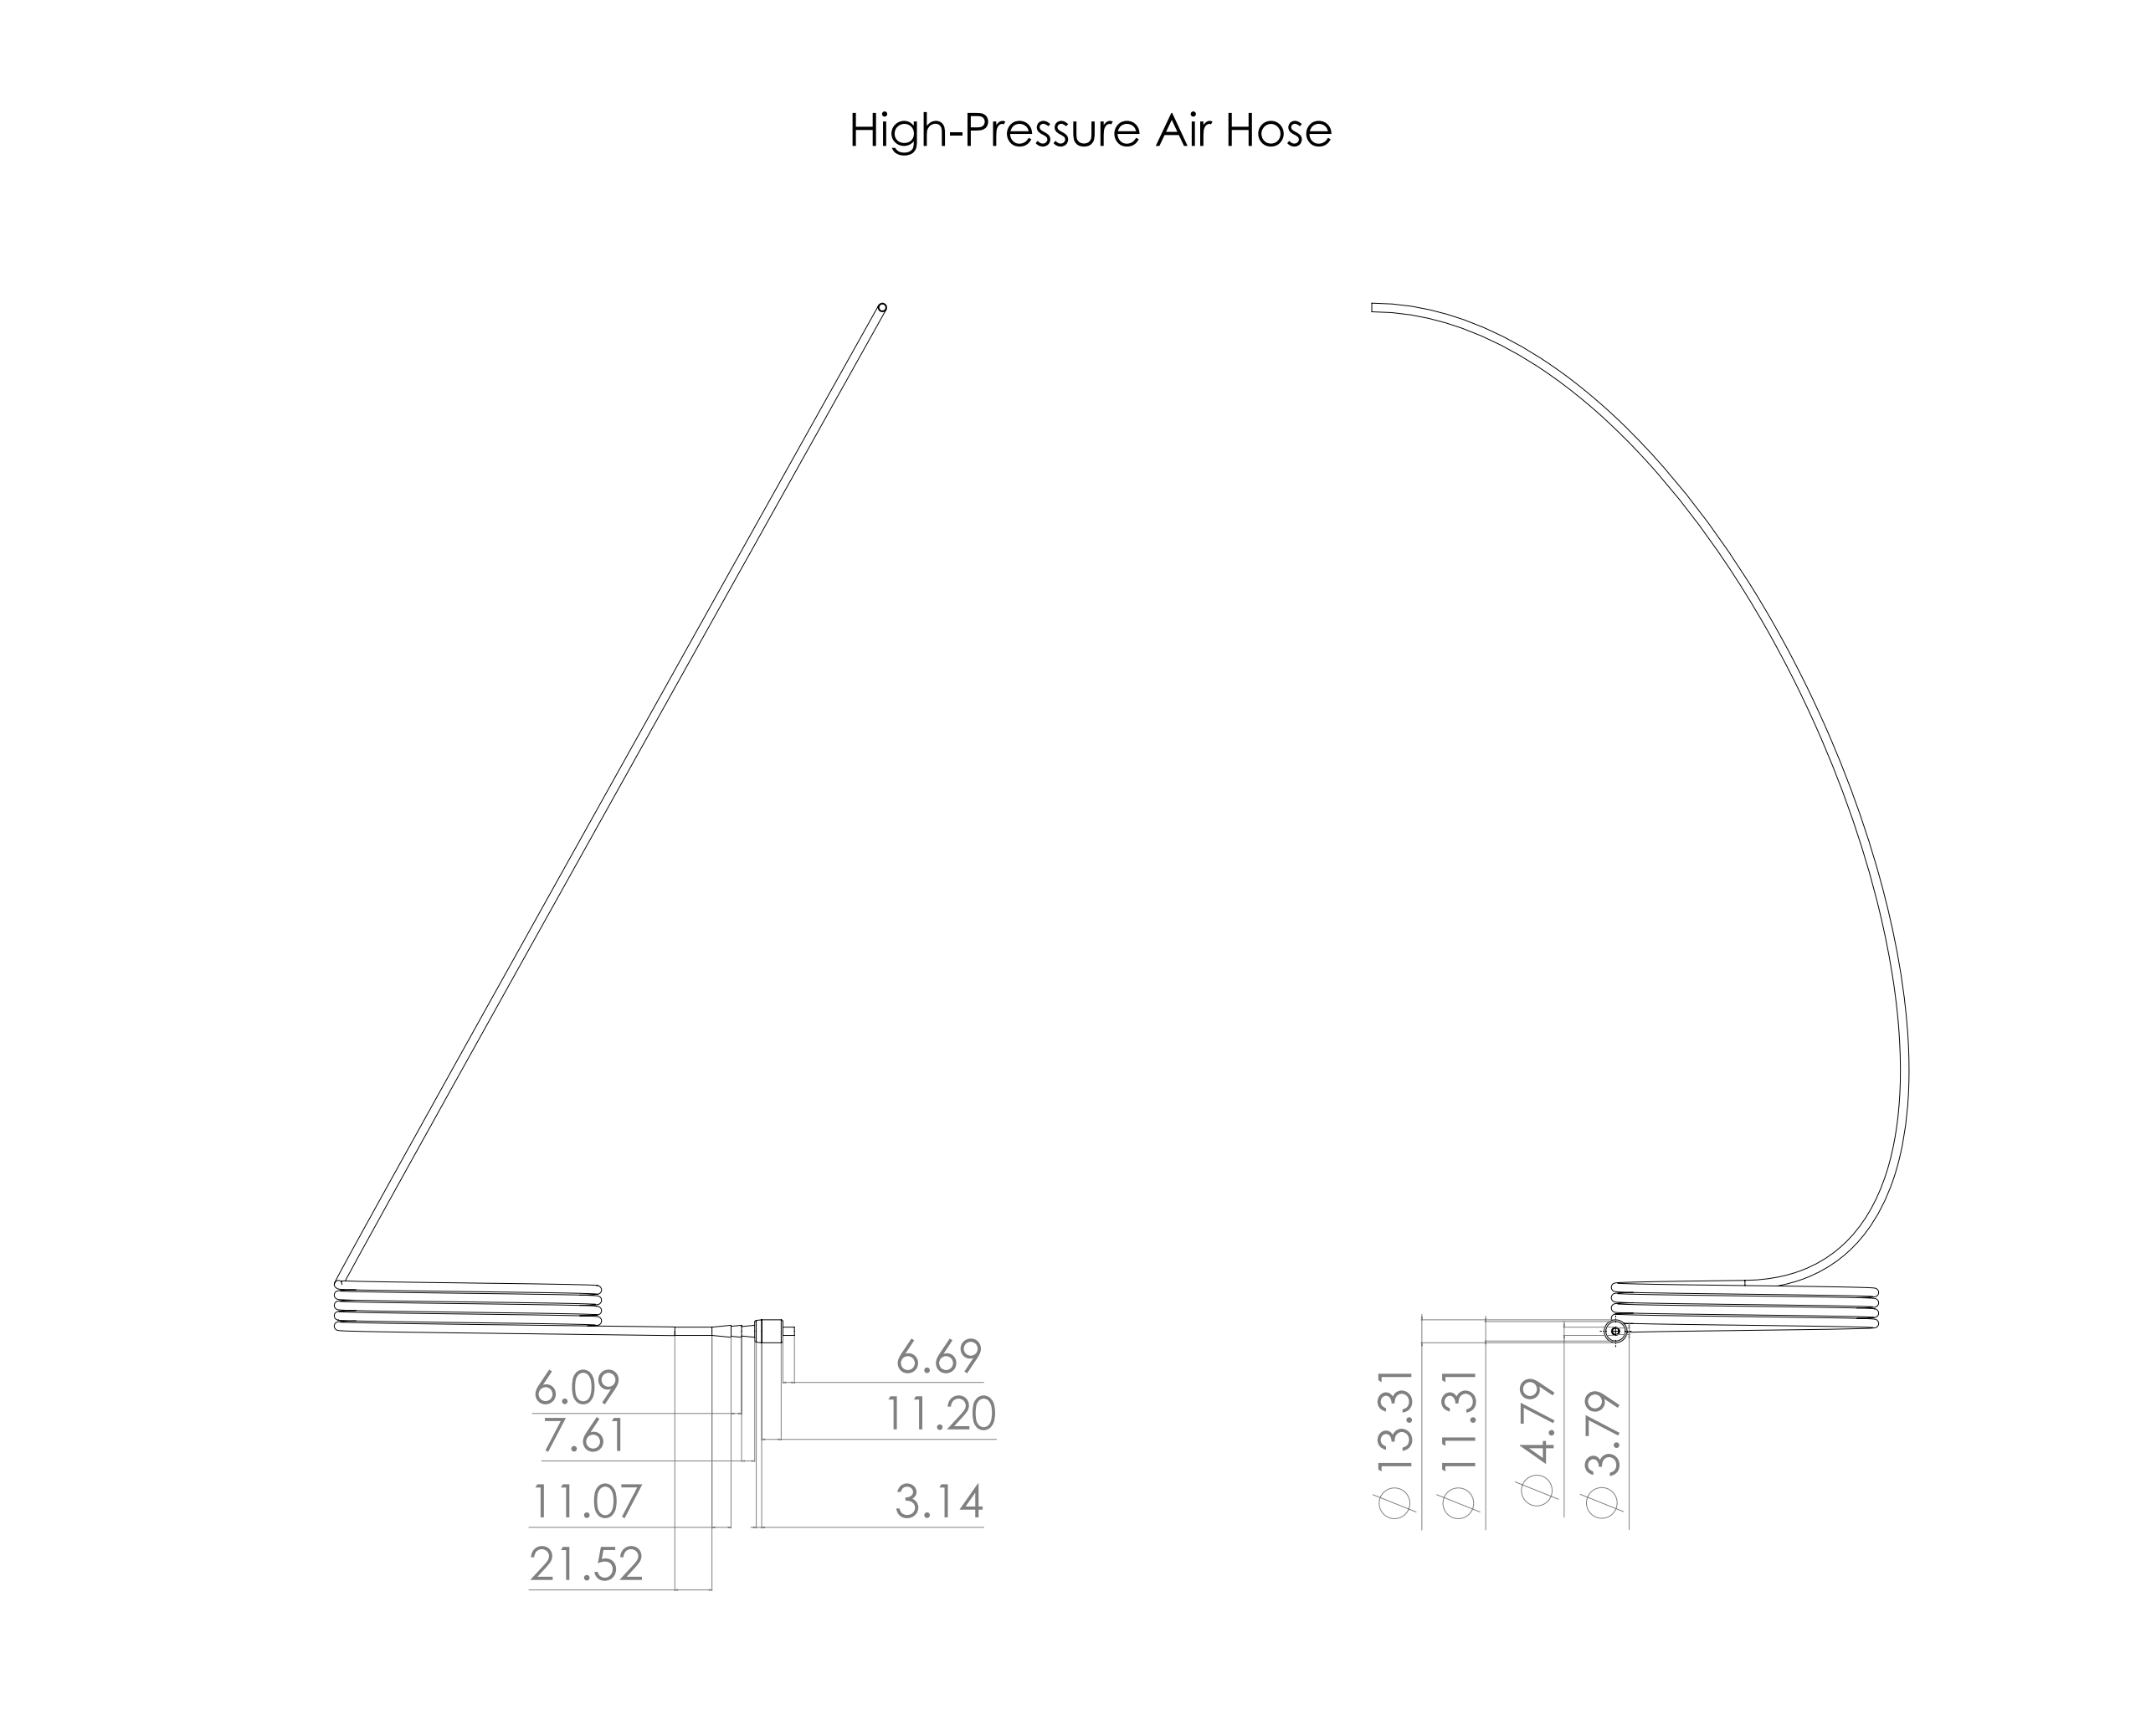
ISO-10303-21;
HEADER;
FILE_DESCRIPTION (('STEP AP214'),
    '1' );
FILE_NAME ('High-Pressure Air Hose.step',
    '2026-10-25T20:52:49',
    ( '' ),
    ( '' ),
    'SwSTEP 2.0',
    'SolidWorks 2025',
    '' );
FILE_SCHEMA (( 'AUTOMOTIVE_DESIGN' ));
ENDSEC;

DATA;
#1=CARTESIAN_POINT ( 'NONE',  ( -113.6132551642233466, -295.8660902273127817, -261.0439986488574391 ) ) ;
#2=CARTESIAN_POINT ( 'NONE',  ( -21.69829453939080111, -272.4952783879842286, -198.0198581616166962 ) ) ;
#3=CARTESIAN_POINT ( 'NONE',  ( -77.14607672046975040, -275.6695791045739270, -333.3258523244866751 ) ) ;
#4=CARTESIAN_POINT ( 'NONE',  ( -96.50722556860337420, -298.4744652489187047, -226.7430298893199279 ) ) ;
#5=CARTESIAN_POINT ( 'NONE',  ( 35.29261755122405475, -294.8217676056252117, -258.4658906454228031 ) ) ;
#7=CARTESIAN_POINT ( 'NONE',  ( 17.20777486049739124, -295.0510334597752831, -319.1340501124739717 ) ) ;
#10=CARTESIAN_POINT ( 'NONE',  ( 23.39288443123379579, -284.9668621146994951, -225.7548735365318748 ) ) ;
#11=CARTESIAN_POINT ( 'NONE',  ( -84.47810206200919936, -295.7221423797171838, -326.1693894271719500 ) ) ;
#12=CARTESIAN_POINT ( 'NONE',  ( -83.27587881292458860, -285.4425543175578923, -208.4961557201596918 ) ) ;
#14=CARTESIAN_POINT ( 'NONE',  ( 24.12276456990134577, -287.8361799259163263, -316.7061702643556487 ) ) ;
#15=CARTESIAN_POINT ( 'NONE',  ( -83.16459577638245548, -297.6555613683490265, -330.2488683299737886 ) ) ;
#16=CARTESIAN_POINT ( 'NONE',  ( 12.16221636192367228, -290.7420802479286976, -214.1725176534357615 ) ) ;
#17=CARTESIAN_POINT ( 'NONE',  ( -48.08606759839130973, -279.1160864900698471, -194.2237662435092886 ) ) ;
#18=CARTESIAN_POINT ( 'NONE',  ( -110.4683760289727132, -293.8380690714490129, -287.0191576251351080 ) ) ;
#20=CARTESIAN_POINT ( 'NONE',  ( 26.72141337091415991, -285.8585362577462661, -234.4374339655554991 ) ) ;
#21=DIRECTION ( 'NONE',  ( -1.000000000000000000, -0.000000000000000000, -0.000000000000000000 ) ) ;
#23=CARTESIAN_POINT ( 'NONE',  ( -111.0120785373717354, -298.2093386174307170, -265.9889607955867632 ) ) ;
#24=CARTESIAN_POINT ( 'NONE',  ( -9.095926160855869469, -281.8396501160608523, -199.3626493647371376 ) ) ;
#25=CARTESIAN_POINT ( 'NONE',  ( -109.2360963732521952, -294.8641011722828580, -247.6139534407837743 ) ) ;
#26=CARTESIAN_POINT ( 'NONE',  ( 24.14595339631129534, -281.7647060850542289, -309.8413200465337241 ) ) ;
#27=CARTESIAN_POINT ( 'NONE',  ( -106.5142501024570265, -297.1531912002984086, -236.5357083837597827 ) ) ;
#29=CARTESIAN_POINT ( 'NONE',  ( -110.4578234273896271, -280.7667899122553763, -253.6568320815989921 ) ) ;
#30=CARTESIAN_POINT ( 'NONE',  ( -93.78727130258138800, -296.2704692607680386, -223.6800016881232693 ) ) ;
#33=CARTESIAN_POINT ( 'NONE',  ( -91.92744132223316456, -285.8159430608695288, -321.2751991526628785 ) ) ;
#35=CARTESIAN_POINT ( 'NONE',  ( -110.4542110544635705, -294.2666405000204577, -253.6410175316879361 ) ) ;
#36=CARTESIAN_POINT ( 'NONE',  ( 16.83410871617971338, -275.5019898621288235, -324.9252248568274126 ) ) ;
#37=CARTESIAN_POINT ( 'NONE',  ( -6.039705354571541562, -292.3087031825515965, -204.3989839164147782 ) ) ;
#38=CARTESIAN_POINT ( 'NONE',  ( 33.63237012736230724, -283.3319559697839054, -290.1951570289018605 ) ) ;
#39=CARTESIAN_POINT ( 'NONE',  ( 33.67317559943808192, -277.4154469211121636, -290.4904342910287482 ) ) ;
#40=CARTESIAN_POINT ( 'NONE',  ( -68.83699650705307249, -285.0594432950156829, -339.7618826965099856 ) ) ;
#41=CARTESIAN_POINT ( 'NONE',  ( 30.69690168102419747, -280.7137460309204471, -297.8907232790041348 ) ) ;
#42=CARTESIAN_POINT ( 'NONE',  ( -110.7162897014109433, -280.3529109521358009, -285.8907753398488580 ) ) ;
#43=CARTESIAN_POINT ( 'NONE',  ( -113.8629036840343218, -272.8260555190163927, -261.7875883216721036 ) ) ;
#44=CARTESIAN_POINT ( 'NONE',  ( 36.88505382238304264, -275.6425748523263906, -290.8892655207978351 ) ) ;
#45=CARTESIAN_POINT ( 'NONE',  ( 22.49833801616120255, -296.0810694518352193, -314.6384715069982576 ) ) ;
#49=CARTESIAN_POINT ( 'NONE',  ( -61.22503046524085590, -293.4984592147682747, -342.3179306570231688 ) ) ;
#50=CARTESIAN_POINT ( 'NONE',  ( -56.87203779738695175, -273.3011920805299724, -199.9055576269083190 ) ) ;
#51=CARTESIAN_POINT ( 'NONE',  ( -39.21425765019228038, -293.5492008878248384, -194.0645109205592576 ) ) ;
#52=CARTESIAN_POINT ( 'NONE',  ( -72.08107566293803359, -300.1233781216987495, -198.2974183793908196 ) ) ;
#53=CARTESIAN_POINT ( 'NONE',  ( -22.28692340252414539, -293.4457659912081908, -195.1980702719413614 ) ) ;
#54=CARTESIAN_POINT ( 'NONE',  ( 17.36828252781073800, -290.2692810089828868, -321.4942518745497182 ) ) ;
#55=CARTESIAN_POINT ( 'NONE',  ( -112.2266234623324124, -276.5486602746883023, -270.6195867653905793 ) ) ;
#56=CARTESIAN_POINT ( 'NONE',  ( -81.65742486183103210, -279.5809590698107172, -330.1727450829594659 ) ) ;
#57=CARTESIAN_POINT ( 'NONE',  ( 35.17272386656721750, -291.8502700334059909, -287.2389789927554489 ) ) ;
#58=CARTESIAN_POINT ( 'NONE',  ( 33.44209198229489743, -283.7601780698271341, -297.3788945958802969 ) ) ;
#59=CARTESIAN_POINT ( 'NONE',  ( -109.8060437348913467, -283.3224215553644285, -281.7842631819470398 ) ) ;
#60=ORIENTED_EDGE ( 'NONE', *, *, #32885, .T. ) ;
#61=CARTESIAN_POINT ( 'NONE',  ( -71.42250952254038054, -283.1821142129608120, -334.9411916729687277 ) ) ;
#62=CARTESIAN_POINT ( 'NONE',  ( -28.27524738754997813, -281.2441658516256098, -194.1546269278096304 ) ) ;
#63=CARTESIAN_POINT ( 'NONE',  ( -113.4234760108877538, -283.4592184142248357, -261.4407986698293485 ) ) ;
#64=CARTESIAN_POINT ( 'NONE',  ( -109.5114376524103363, -279.1602184646021101, -296.6766189074363638 ) ) ;
#66=CARTESIAN_POINT ( 'NONE',  ( -97.37137399137552052, -279.4367685291730368, -317.4689306191668265 ) ) ;
#68=CARTESIAN_POINT ( 'NONE',  ( -6.941161984400275209, -297.1233781216987495, -333.4151289067050357 ) ) ;
#71=CARTESIAN_POINT ( 'NONE',  ( -93.35509533216730915, -299.2464325822394926, -220.4862725388631191 ) ) ;
#73=CARTESIAN_POINT ( 'NONE',  ( -88.23497865206087454, -275.7892183208580263, -324.9662551183911319 ) ) ;
#74=CARTESIAN_POINT ( 'NONE',  ( -102.3605472477040337, -292.8335325276641470, -230.9337581368000087 ) ) ;
#75=CARTESIAN_POINT ( 'NONE',  ( 34.31805428248770795, -292.7103970009527529, -255.9121641687935949 ) ) ;
#76=CARTESIAN_POINT ( 'NONE',  ( -96.34789938153127764, -289.3946153186523702, -319.7555901667715261 ) ) ;
#78=CARTESIAN_POINT ( 'NONE',  ( 36.88326735793300060, -292.3562425583122035, -288.5613484753777129 ) ) ;
#79=CARTESIAN_POINT ( 'NONE',  ( -33.17331374697837987, -284.5052435883285966, -196.6285636872405860 ) ) ;
#80=CARTESIAN_POINT ( 'NONE',  ( -69.57500681174269630, -293.4837748164715094, -203.4749671060159528 ) ) ;
#81=CARTESIAN_POINT ( 'NONE',  ( 22.22138339417639230, -283.4657779623778993, -313.4347628960813381 ) ) ;
#82=CARTESIAN_POINT ( 'NONE',  ( -28.99082608718071796, -289.8901462222868872, -346.7236095928074064 ) ) ;
#83=CARTESIAN_POINT ( 'NONE',  ( 34.39346676443356188, -281.8609718709653862, -256.4368729998031426 ) ) ;
#84=CARTESIAN_POINT ( 'NONE',  ( 39.20951696572362977, -292.3824562929385706, -273.1753459359540557 ) ) ;
#85=CARTESIAN_POINT ( 'NONE',  ( -4.393016225146153531, -289.4317384794202326, -339.7912944455955540 ) ) ;
#86=CARTESIAN_POINT ( 'NONE',  ( 37.65823291392757000, -287.8290301222977519, -253.1405899415904912 ) ) ;
#87=CARTESIAN_POINT ( 'NONE',  ( -52.09100773288315622, -286.0247242745892322, -198.8666571505329728 ) ) ;
#90=CARTESIAN_POINT ( 'NONE',  ( 3.580403759654407825, -296.3688474698320192, -334.1856371305267430 ) ) ;
#91=CARTESIAN_POINT ( 'NONE',  ( -113.1662103178394432, -295.1037629167083196, -280.9449385996212527 ) ) ;
#93=CARTESIAN_POINT ( 'NONE',  ( -83.57703501779413102, -278.4588845934780466, -213.5002235206053740 ) ) ;
#94=CARTESIAN_POINT ( 'NONE',  ( -113.8008141857499993, -272.1671345119243028, -261.7861089057840900 ) ) ;
#95=CARTESIAN_POINT ( 'NONE',  ( -103.3981541237931054, -294.5919941891141889, -303.1453271309203501 ) ) ;
#96=CARTESIAN_POINT ( 'NONE',  ( 35.36480375133581333, -277.1321324331269693, -256.5141577024394337 ) ) ;
#97=CARTESIAN_POINT ( 'NONE',  ( -54.47399014668751249, -271.9692736385993044, -198.1298912440302331 ) ) ;
#98=CARTESIAN_POINT ( 'NONE',  ( 29.09142378860511258, -294.3365518058123484, -239.0359238687793777 ) ) ;
#99=CARTESIAN_POINT ( 'NONE',  ( -75.80859898051943446, -296.6581450815154994, -332.8264140846681016 ) ) ;
#101=CARTESIAN_POINT ( 'NONE',  ( -85.24696079806301441, -293.7120025854050596, -328.2844675371921994 ) ) ;
#102=CARTESIAN_POINT ( 'NONE',  ( -114.1802237732302245, -273.3548555386022372, -270.3713173946429720 ) ) ;
#103=CARTESIAN_POINT ( 'NONE',  ( -94.45286519521168600, -275.2254758110098010, -221.7273418318577569 ) ) ;
#104=CARTESIAN_POINT ( 'NONE',  ( -108.8900272069156472, -291.2871953198740016, -286.0477213144812936 ) ) ;
#105=CARTESIAN_POINT ( 'NONE',  ( -4.323302397459051427, -294.9377782480969472, -335.5047827706411567 ) ) ;
#106=CARTESIAN_POINT ( 'NONE',  ( -112.5882073356291926, -280.4803416563776182, -274.4070978670125669 ) ) ;
#107=CARTESIAN_POINT ( 'NONE',  ( -108.0504587551557307, -277.6107128976585159, -241.1452023711554489 ) ) ;
#108=CARTESIAN_POINT ( 'NONE',  ( -33.07270939256004993, -282.3483276930217585, -347.1537153405075173 ) ) ;
#109=CARTESIAN_POINT ( 'NONE',  ( 15.96235870874075324, -274.1327303341880679, -214.9355814682232904 ) ) ;
#110=CARTESIAN_POINT ( 'NONE',  ( -96.18649800141388084, -277.6093990147008412, -221.9287466249451199 ) ) ;
#111=CARTESIAN_POINT ( 'NONE',  ( -61.43528157839729431, -277.7399057781236706, -199.1056149990290294 ) ) ;
#112=CARTESIAN_POINT ( 'NONE',  ( -67.00311722930408109, -296.3398741006864157, -203.1056652694137199 ) ) ;
#113=CARTESIAN_POINT ( 'NONE',  ( -33.55588428573118165, -276.0999399286864104, -195.4440965705611575 ) ) ;
#115=CARTESIAN_POINT ( 'NONE',  ( 5.580496127948171292, -290.6504686268311843, -208.4249260671794843 ) ) ;
#116=CARTESIAN_POINT ( 'NONE',  ( -112.2626902172997205, -290.3291827781827692, -288.1895695498705550 ) ) ;
#117=CARTESIAN_POINT ( 'NONE',  ( -66.84020672111827821, -275.6666780896798059, -201.2245391158463406 ) ) ;
#118=CARTESIAN_POINT ( 'NONE',  ( -41.95658063400141202, -295.9936855060223024, -195.6702128762018162 ) ) ;
#119=CARTESIAN_POINT ( 'NONE',  ( -106.5292690430238025, -284.1790909977862043, -236.9359907930603981 ) ) ;
#120=CARTESIAN_POINT ( 'NONE',  ( -37.35456021389456538, -284.0517986001094073, -195.3485413134038424 ) ) ;
#122=CARTESIAN_POINT ( 'NONE',  ( 17.04267055929170738, -291.6439787220554649, -220.9968955086508515 ) ) ;
#123=CARTESIAN_POINT ( 'NONE',  ( -62.96739064857778345, -283.8546313715036717, -200.6342915240590230 ) ) ;
#126=CARTESIAN_POINT ( 'NONE',  ( 7.902484555432940816, -290.6701741179288092, -210.5450298619024636 ) ) ;
#127=CARTESIAN_POINT ( 'NONE',  ( -89.97405692109779807, -282.2588973123018832, -325.6834086931719412 ) ) ;
#128=CARTESIAN_POINT ( 'NONE',  ( -103.8431496891660544, -279.7226268398578668, -302.4792602913342421 ) ) ;
#129=CARTESIAN_POINT ( 'NONE',  ( -65.74447246362868214, -286.8938844950662883, -199.2042825010933313 ) ) ;
#130=CARTESIAN_POINT ( 'NONE',  ( -9.493390062269362772, -286.4264726012228266, -202.8681937675485756 ) ) ;
#131=CARTESIAN_POINT ( 'NONE',  ( -94.04857214285830480, -279.3176295112319281, -317.2818740737955068 ) ) ;
#132=CARTESIAN_POINT ( 'NONE',  ( -94.07220428401220147, -280.0074554778488505, -224.1631567100062625 ) ) ;
#134=CARTESIAN_POINT ( 'NONE',  ( -96.45200547131824464, -285.9190198393021092, -316.5235751886017397 ) ) ;
#136=CARTESIAN_POINT ( 'NONE',  ( -46.12776598691637275, -297.7769461629130774, -193.8640261997899188 ) ) ;
#138=CARTESIAN_POINT ( 'NONE',  ( -23.45499506039496396, -290.8538007153030662, -343.7556936576084468 ) ) ;
#141=CARTESIAN_POINT ( 'NONE',  ( -72.02372285203398405, -285.9805209788416391, -342.4524372437778652 ) ) ;
#143=CARTESIAN_POINT ( 'NONE',  ( 35.52797234631308498, -291.6693239864514453, -248.0799319934128278 ) ) ;
#144=CARTESIAN_POINT ( 'NONE',  ( -9.246811333089969054, -287.9463490696106192, -202.2197728238365926 ) ) ;
#145=CARTESIAN_POINT ( 'NONE',  ( 34.64086854919326441, -283.5370289157921775, -287.6338091762179943 ) ) ;
#146=CARTESIAN_POINT ( 'NONE',  ( 23.68266680496880738, -289.5944490205463921, -316.3462561790806831 ) ) ;
#147=CARTESIAN_POINT ( 'NONE',  ( -5.814316714654535367, -289.9613947498637572, -340.0699579485100230 ) ) ;
#148=CARTESIAN_POINT ( 'NONE',  ( -108.8862810617042669, -286.2619989188776231, -292.8638642162096630 ) ) ;
#149=CARTESIAN_POINT ( 'NONE',  ( -111.7315784639272209, -278.9682992199453224, -250.4319288396881689 ) ) ;
#151=CARTESIAN_POINT ( 'NONE',  ( 37.80224029141654540, -291.7390338754980235, -278.7595689655631759 ) ) ;
#152=CARTESIAN_POINT ( 'NONE',  ( 36.17633980381252456, -281.0978762120507781, -247.4679353929731462 ) ) ;
#153=CARTESIAN_POINT ( 'NONE',  ( -66.31674629447961422, -275.5291285280121656, -202.0141196464570328 ) ) ;
#155=CARTESIAN_POINT ( 'NONE',  ( -20.25526795762937127, -294.7662352645559167, -195.3538533559490702 ) ) ;
#156=CARTESIAN_POINT ( 'NONE',  ( -41.11966117830017708, -272.2452171050537686, -194.4168510268810053 ) ) ;
#158=CARTESIAN_POINT ( 'NONE',  ( -95.65708358510205755, -278.6778134938541598, -226.3255324265030310 ) ) ;
#159=CARTESIAN_POINT ( 'NONE',  ( 38.33293935469181690, -276.6066984866882876, -258.3872807340205213 ) ) ;
#160=CARTESIAN_POINT ( 'NONE',  ( -35.81830170358009724, -299.4968625532499118, -196.7715064960510745 ) ) ;
#161=CARTESIAN_POINT ( 'NONE',  ( -70.37975053163600592, -282.5357189658061543, -339.6670035245268764 ) ) ;
#162=CARTESIAN_POINT ( 'NONE',  ( -108.6968154583750703, -292.0538962897698525, -290.2073774136056272 ) ) ;
#163=CARTESIAN_POINT ( 'NONE',  ( -35.86450529380874741, -299.5904438321611565, -194.0540724790644447 ) ) ;
#164=CARTESIAN_POINT ( 'NONE',  ( -110.4388770307767373, -298.0485552961351345, -247.2764033145294036 ) ) ;
#165=CARTESIAN_POINT ( 'NONE',  ( -15.02233590537950114, -296.7627049945999715, -341.8430372460552462 ) ) ;
#166=CARTESIAN_POINT ( 'NONE',  ( -104.6730707308207968, -282.1193390125066003, -303.1377496322695038 ) ) ;
#167=CARTESIAN_POINT ( 'NONE',  ( -113.9853605009663795, -290.3155259493814242, -262.6348601863189174 ) ) ;
#168=CARTESIAN_POINT ( 'NONE',  ( -79.76971251359887560, -271.4959503811738273, -208.8840916564036263 ) ) ;
#169=CARTESIAN_POINT ( 'NONE',  ( 2.307177052818977447, -288.1741521440539486, -205.2887970377841498 ) ) ;
#170=CARTESIAN_POINT ( 'NONE',  ( -108.0463951965091098, -289.7272753538697998, -250.9943379319703922 ) ) ;
#171=CARTESIAN_POINT ( 'NONE',  ( 201.3067182052938051, 288.2280244914530840, -97.39779909378675882 ) ) ;
#173=CARTESIAN_POINT ( 'NONE',  ( -109.8658504693686382, -289.4339475807516351, -246.1362763784779304 ) ) ;
#174=CARTESIAN_POINT ( 'NONE',  ( -5.787136446112612020, -288.2921266566153236, -336.2124429329496706 ) ) ;
#176=CARTESIAN_POINT ( 'NONE',  ( -100.7487074920235273, -286.2040526672859073, -227.1274661871449609 ) ) ;
#177=CARTESIAN_POINT ( 'NONE',  ( -69.25682644265404520, -277.8172129950345379, -336.0522927072145194 ) ) ;
#178=CARTESIAN_POINT ( 'NONE',  ( 36.06976937112843729, -292.7541342344004534, -292.7275812612277264 ) ) ;
#179=CARTESIAN_POINT ( 'NONE',  ( -38.72238868582785898, -283.7204533004693872, -347.2467895094548567 ) ) ;
#180=CARTESIAN_POINT ( 'NONE',  ( -10.92373924738846114, -284.2341409807796140, -342.0049621938744622 ) ) ;
#181=CARTESIAN_POINT ( 'NONE',  ( -94.38063292225054113, -284.1828072836642036, -322.0750035236984559 ) ) ;
#182=CARTESIAN_POINT ( 'NONE',  ( 28.99011267871087938, -281.4722031727284275, -239.7083648369550417 ) ) ;
#183=CARTESIAN_POINT ( 'NONE',  ( 180.6301689436333788, 254.0011452960685006, -166.8208226387889113 ) ) ;
#184=CARTESIAN_POINT ( 'NONE',  ( 196.3077706885435134, 285.2721524738067274, -111.5570765633820969 ) ) ;
#185=CARTESIAN_POINT ( 'NONE',  ( -90.09665665672530110, -228.8726286412962736, -344.7822526990161691 ) ) ;
#186=CARTESIAN_POINT ( 'NONE',  ( -69.55286334857535735, -272.8140695680438057, -204.6721334301478521 ) ) ;
#187=CARTESIAN_POINT ( 'NONE',  ( -11.36788948023329482, -273.3188565473291192, -201.7533031230518077 ) ) ;
#188=CARTESIAN_POINT ( 'NONE',  ( -68.20725116294569546, -294.9544458090643957, -340.8369625160823375 ) ) ;
#189=CARTESIAN_POINT ( 'NONE',  ( 6.867305562803349694, -59.82436178187390396, -351.3599612539230748 ) ) ;
#190=CARTESIAN_POINT ( 'NONE',  ( -66.02668222974523360, -272.3693846100331939, -199.4212332350789154 ) ) ;
#191=CARTESIAN_POINT ( 'NONE',  ( -37.17015063146384790, -299.9147455406174458, -196.1229585654807863 ) ) ;
#192=CARTESIAN_POINT ( 'NONE',  ( 19.90811401000262038, -289.5144666564462455, -316.4447621617657092 ) ) ;
#194=CARTESIAN_POINT ( 'NONE',  ( -70.69477044455324233, -296.4224833217160153, -339.5159684217153426 ) ) ;
#195=CARTESIAN_POINT ( 'NONE',  ( 17.81853407656373633, -287.3620640795646182, -222.4514425058484051 ) ) ;
#196=CARTESIAN_POINT ( 'NONE',  ( -58.02497702157741344, -272.7114924129007250, -196.4567845684104839 ) ) ;
#197=CARTESIAN_POINT ( 'NONE',  ( 36.21809064911852261, -294.6363344162023736, -292.7476569483883964 ) ) ;
#198=CARTESIAN_POINT ( 'NONE',  ( -104.5460947458797278, -296.5572545471907802, -307.9279408047181050 ) ) ;
#199=CARTESIAN_POINT ( 'NONE',  ( -110.3370228416248295, -290.7079322884769113, -271.1874753075676949 ) ) ;
#201=CARTESIAN_POINT ( 'NONE',  ( -69.54077655466207375, -275.5518863169126007, -201.9910387382556678 ) ) ;
#202=CARTESIAN_POINT ( 'NONE',  ( 38.34100351736458379, -274.5000774477773575, -282.5315648924769221 ) ) ;
#205=CARTESIAN_POINT ( 'NONE',  ( -104.9245238535658160, -277.5835944543852634, -307.1318786540637120 ) ) ;
#207=CARTESIAN_POINT ( 'NONE',  ( 31.87562710300615620, -273.6143523044818266, -244.7602971938240444 ) ) ;
#208=CARTESIAN_POINT ( 'NONE',  ( -108.8394098029810380, -273.8445740299966928, -254.1653288387956025 ) ) ;
#209=CARTESIAN_POINT ( 'NONE',  ( -1.618296635492913360, -275.4792631490921053, -206.4151797416647582 ) ) ;
#210=CARTESIAN_POINT ( 'NONE',  ( -31.36245263867117217, -275.8867941206686396, -194.5969546141441526 ) ) ;
#212=CARTESIAN_POINT ( 'NONE',  ( 20.45256449681794564, -274.2372513224178761, -318.7163636411478933 ) ) ;
#213=CARTESIAN_POINT ( 'NONE',  ( -26.18367686562210039, -295.5577560403836515, -342.6064720533350396 ) ) ;
#214=CARTESIAN_POINT ( 'NONE',  ( 35.49350546835615461, -291.9893731014084892, -259.8536090943885597 ) ) ;
#216=CARTESIAN_POINT ( 'NONE',  ( -102.0418390638001398, -278.4966892230997360, -312.0926700045682196 ) ) ;
#217=CARTESIAN_POINT ( 'NONE',  ( 34.12090894609900005, -275.5214342262589753, -255.3972326369435280 ) ) ;
#218=CARTESIAN_POINT ( 'NONE',  ( -26.67319746492361787, -284.8698424366841664, -194.5485961385973042 ) ) ;
#219=CARTESIAN_POINT ( 'NONE',  ( -69.98802764187368552, -297.4812203234077970, -338.0823389745905843 ) ) ;
#221=CARTESIAN_POINT ( 'NONE',  ( -95.07820106282620998, -284.3812749118341685, -225.4064025234517032 ) ) ;
#222=CARTESIAN_POINT ( 'NONE',  ( -62.15031415579434082, -275.6189368971078579, -340.1472874860159550 ) ) ;
#223=CARTESIAN_POINT ( 'NONE',  ( -95.75169594866139278, -276.5021968402988364, -315.1232370903478568 ) ) ;
#224=CARTESIAN_POINT ( 'NONE',  ( -110.1547686304307092, -286.7838384147241300, -252.3291687126599356 ) ) ;
#225=CARTESIAN_POINT ( 'NONE',  ( 5.641680306182056626, -277.6606581397782065, -329.9180858645652279 ) ) ;
#227=CARTESIAN_POINT ( 'NONE',  ( 16.37664934189118426, -274.7048225403960942, -324.4790114041376796 ) ) ;
#228=CARTESIAN_POINT ( 'NONE',  ( 34.80913351221764174, -276.3624349405349108, -282.4209052261880402 ) ) ;
#229=CARTESIAN_POINT ( 'NONE',  ( 2.820361398021606458, -282.5894332162787350, -206.7619648397659091 ) ) ;
#231=CARTESIAN_POINT ( 'NONE',  ( 34.47262405957937403, -289.1691442991094618, -246.6989133634617701 ) ) ;
#232=CARTESIAN_POINT ( 'NONE',  ( 21.86556464674976041, -292.1835024172012822, -316.4195789663704090 ) ) ;
#234=CARTESIAN_POINT ( 'NONE',  ( -41.87763380309878869, -296.7886418773014725, -197.1043380165232293 ) ) ;
#235=CARTESIAN_POINT ( 'NONE',  ( -106.8591441079072695, -289.0350993510990065, -244.1732922129692724 ) ) ;
#236=CARTESIAN_POINT ( 'NONE',  ( -114.4693268140674434, -273.6886850827510216, -284.2063049943780015 ) ) ;
#238=CARTESIAN_POINT ( 'NONE',  ( -23.45726847500185741, -287.3577760870506950, -345.4476048667748955 ) ) ;
#239=CARTESIAN_POINT ( 'NONE',  ( -33.75247087138109237, -284.3366009130915018, -194.4592639308252728 ) ) ;
#240=CARTESIAN_POINT ( 'NONE',  ( -78.69286312455705001, -285.0466963355058851, -331.2335767372052260 ) ) ;
#241=CARTESIAN_POINT ( 'NONE',  ( -107.9142151825760436, -285.1001298097412473, -289.6988518128527517 ) ) ;
#242=CARTESIAN_POINT ( 'NONE',  ( -50.30864909105871163, -293.8672956765573758, -196.1299585228881313 ) ) ;
#243=CARTESIAN_POINT ( 'NONE',  ( -66.22322631712503949, -274.0175736708989689, -198.9914908511120188 ) ) ;
#244=CARTESIAN_POINT ( 'NONE',  ( -82.02121176197549346, -287.7358496163018913, -331.2959638059363101 ) ) ;
#245=CARTESIAN_POINT ( 'NONE',  ( -99.64976321348814281, -277.9516674045289619, -315.6240650913662762 ) ) ;
#246=CARTESIAN_POINT ( 'NONE',  ( 31.35993196141822281, -295.1472400932031519, -241.0411030402186157 ) ) ;
#248=CARTESIAN_POINT ( 'NONE',  ( 35.78497577281001440, -296.2662352645559167, -287.0191576251351080 ) ) ;
#249=CARTESIAN_POINT ( 'NONE',  ( -18.62610965303630906, -281.4909754024122890, -341.4840500770574181 ) ) ;
#251=CARTESIAN_POINT ( 'NONE',  ( -39.50340962879238305, -278.0248805946041557, -195.3795613189264202 ) ) ;
#253=CARTESIAN_POINT ( 'NONE',  ( -97.25653598327876637, -271.6698244868129564, -223.1073329477313791 ) ) ;
#254=CARTESIAN_POINT ( 'NONE',  ( 34.47519203589411774, -274.7209678462776878, -256.7146287507716806 ) ) ;
#255=CARTESIAN_POINT ( 'NONE',  ( -0.9307921106466295891, -294.0650048284701370, -206.2765958823960943 ) ) ;
#256=CARTESIAN_POINT ( 'NONE',  ( 34.55765642826714412, -294.6765038290132566, -284.2855919575040389 ) ) ;
#257=CARTESIAN_POINT ( 'NONE',  ( 37.74284114224520437, -294.7987799472403481, -256.1865648562181832 ) ) ;
#258=CARTESIAN_POINT ( 'NONE',  ( 37.27658265588780040, -294.6540076195757933, -253.4083519683468353 ) ) ;
#259=CARTESIAN_POINT ( 'NONE',  ( -108.8851482201205414, -296.1932415551128202, -284.9332040079801800 ) ) ;
#260=CARTESIAN_POINT ( 'NONE',  ( -111.3897608342564070, -292.3983347659790866, -282.3532917929296673 ) ) ;
#261=CARTESIAN_POINT ( 'NONE',  ( -41.56701483115121221, -283.2705272460136712, -347.2974267954927541 ) ) ;
#262=CARTESIAN_POINT ( 'NONE',  ( -18.82848769330092153, -272.4274859315958111, -196.8388344709858018 ) ) ;
#263=CARTESIAN_POINT ( 'NONE',  ( 22.99321104538541860, -286.7450741532542224, -222.4997577815586851 ) ) ;
#264=CARTESIAN_POINT ( 'NONE',  ( -92.15899064099502880, -279.8196800380848686, -321.1009690803662124 ) ) ;
#265=CARTESIAN_POINT ( 'NONE',  ( -8.150179586038067470, -285.5028795466129736, -203.1951773795938152 ) ) ;
#267=CARTESIAN_POINT ( 'NONE',  ( -77.09840566266530004, -287.5843468112212804, -334.0173477355417617 ) ) ;
#268=CARTESIAN_POINT ( 'NONE',  ( -45.12257076738355721, -278.0943342815326105, -194.9447721771423971 ) ) ;
#269=CARTESIAN_POINT ( 'NONE',  ( -107.8893720497363518, -252.3744610414916565, -325.2219058921743908 ) ) ;
#271=CARTESIAN_POINT ( 'NONE',  ( -103.0707657646160413, -283.6269096832978107, -302.3783997235955212 ) ) ;
#273=CARTESIAN_POINT ( 'NONE',  ( 37.16576817676342159, -282.9815768181842373, -288.2116639322431979 ) ) ;
#274=CARTESIAN_POINT ( 'NONE',  ( -4.444799110440903256, -287.6879362380452108, -339.7341427214811347 ) ) ;
#275=CARTESIAN_POINT ( 'NONE',  ( -111.3928543446432258, -279.9245025573324597, -288.3842106415503395 ) ) ;
#276=CARTESIAN_POINT ( 'NONE',  ( -48.40600831671226700, -278.5052016875781078, -346.1172373858461242 ) ) ;
#277=CARTESIAN_POINT ( 'NONE',  ( -92.20703582126834874, -279.0729676217148949, -222.1882355758204994 ) ) ;
#278=CARTESIAN_POINT ( 'NONE',  ( -79.81114824688718556, -275.4550972370517457, -208.9127111854542704 ) ) ;
#279=CARTESIAN_POINT ( 'NONE',  ( 33.32439624573670045, -293.1624354433766939, -239.7783969903679804 ) ) ;
#280=CARTESIAN_POINT ( 'NONE',  ( -23.50445829584242219, -286.8946535863967711, -343.7650351519840797 ) ) ;
#282=CARTESIAN_POINT ( 'NONE',  ( -70.56748717621604783, -293.2214596486516598, -201.7864324643425675 ) ) ;
#283=CARTESIAN_POINT ( 'NONE',  ( -108.4715376898812877, -295.7062291228027675, -252.5679424721457451 ) ) ;
#284=CARTESIAN_POINT ( 'NONE',  ( -15.59057583108496203, -294.4296390795713592, -340.1206596468418297 ) ) ;
#285=CARTESIAN_POINT ( 'NONE',  ( -77.02114960951715261, -292.6137018445027707, -204.6718712135360647 ) ) ;
#286=CARTESIAN_POINT ( 'NONE',  ( 7.197872772093760751, -281.3285238675737787, -212.3305421225269640 ) ) ;
#287=CARTESIAN_POINT ( 'NONE',  ( -31.92281438307887598, -297.0388370913102563, -193.6711941998320015 ) ) ;
#288=CARTESIAN_POINT ( 'NONE',  ( -105.0622752010226577, -290.7319065036531924, -306.7923751401537515 ) ) ;
#289=CARTESIAN_POINT ( 'NONE',  ( -87.52147800885803974, -281.8828391876222099, -327.1964541124606853 ) ) ;
#290=CARTESIAN_POINT ( 'NONE',  ( -114.1670047289575791, -290.9462267493518084, -265.5013994278262999 ) ) ;
#292=CARTESIAN_POINT ( 'NONE',  ( -17.17010717937488096, -286.6529688014165345, -200.1285271177430332 ) ) ;
#294=CARTESIAN_POINT ( 'NONE',  ( -113.9112430796897115, -271.1015500560408213, -283.8576724739366455 ) ) ;
#295=CARTESIAN_POINT ( 'NONE',  ( -39.22682415819677715, -139.9825792601168644, -360.8488084492784083 ) ) ;
#296=CARTESIAN_POINT ( 'NONE',  ( -94.91159530925413890, -278.3846945089381961, -225.1933234040334071 ) ) ;
#297=CARTESIAN_POINT ( 'NONE',  ( -67.42059858149401919, -278.5684387154228716, -203.4932414482983347 ) ) ;
#298=CARTESIAN_POINT ( 'NONE',  ( 18.07732448069620190, -274.4864427186229250, -216.8572984162106252 ) ) ;
#299=CARTESIAN_POINT ( 'NONE',  ( -92.64007872224544826, -240.2551808938772240, -339.7428190326851905 ) ) ;
#300=CARTESIAN_POINT ( 'NONE',  ( -95.44584374818370520, -277.8015992959548726, -220.7172953016149393 ) ) ;
#301=CARTESIAN_POINT ( 'NONE',  ( -68.49327023195247932, -281.4836232829917435, -338.1949331952813509 ) ) ;
#302=CARTESIAN_POINT ( 'NONE',  ( 10.57689206411022553, -296.1611599144177376, -329.4016677618776612 ) ) ;
#303=CARTESIAN_POINT ( 'NONE',  ( -37.55642042354166676, -292.5417769992668582, -197.2874406787996691 ) ) ;
#304=CARTESIAN_POINT ( 'NONE',  ( 23.91132114415732346, -286.7970199167970122, -310.9958052702095870 ) ) ;
#305=CARTESIAN_POINT ( 'NONE',  ( 25.23911174490946863, -275.6105727896177768, -225.6512951641706479 ) ) ;
#306=CARTESIAN_POINT ( 'NONE',  ( -91.84630622800007416, -297.4132482821498797, -221.7993231391932341 ) ) ;
#310=CARTESIAN_POINT ( 'NONE',  ( -50.70934710825899572, -281.8028321744117193, -195.9929782340904580 ) ) ;
#311=CARTESIAN_POINT ( 'NONE',  ( -27.53056093681999172, -281.2592550515166749, -197.6600890250774967 ) ) ;
#312=CARTESIAN_POINT ( 'NONE',  ( -31.17860052041886831, -281.8889978174094040, -194.5728002490756694 ) ) ;
#313=CARTESIAN_POINT ( 'NONE',  ( -5.942905713229805542, -281.6877908578424581, -336.5377726664386273 ) ) ;
#314=CARTESIAN_POINT ( 'NONE',  ( 21.24440329897678836, -273.4090717797046182, -225.6371385638898062 ) ) ;
#317=CARTESIAN_POINT ( 'NONE',  ( 28.96178146475818593, -276.8614997905642667, -309.1941857057189509 ) ) ;
#319=CARTESIAN_POINT ( 'NONE',  ( 4.769913331632007036, -278.4835506822664115, -332.4224800237890918 ) ) ;
#320=CARTESIAN_POINT ( 'NONE',  ( -39.96107325075033145, -275.6591585686044255, -346.7399479336539230 ) ) ;
#323=CARTESIAN_POINT ( 'NONE',  ( -52.56024909002068313, -285.2259183838634158, -344.2168985579138507 ) ) ;
#324=CARTESIAN_POINT ( 'NONE',  ( 28.53551074124957410, -293.1804526957525354, -302.3023540898434476 ) ) ;
#325=CARTESIAN_POINT ( 'NONE',  ( 26.27770430026630777, -286.3302106616349647, -227.1417106107467703 ) ) ;
#326=CARTESIAN_POINT ( 'NONE',  ( -87.63360837066642262, -282.0053727907281882, -324.7331695838644805 ) ) ;
#327=CARTESIAN_POINT ( 'NONE',  ( -34.84458204204858589, -281.5949315533735557, -343.9205063545541066 ) ) ;
#328=CARTESIAN_POINT ( 'NONE',  ( 25.90896429186087957, -283.2670875563693471, -307.6971038925671564 ) ) ;
#329=CARTESIAN_POINT ( 'NONE',  ( -24.47694389544438565, -272.2160532552937866, -196.4199350418342647 ) ) ;
#331=CARTESIAN_POINT ( 'NONE',  ( -110.7265842235424458, -282.6921952033420098, -290.8818197932454837 ) ) ;
#332=CARTESIAN_POINT ( 'NONE',  ( -58.26820715863784272, -297.3226295211096044, -342.4366403366163922 ) ) ;
#334=CARTESIAN_POINT ( 'NONE',  ( -85.64834529566002175, -280.3052127297970628, -215.3168041969837248 ) ) ;
#335=CARTESIAN_POINT ( 'NONE',  ( -5.572524851392624434, -288.4691924952029467, -202.2380827223223321 ) ) ;
#338=CARTESIAN_POINT ( 'NONE',  ( 23.63759464484336092, -294.8685903048981345, -225.7422900162428050 ) ) ;
#340=CARTESIAN_POINT ( 'NONE',  ( -39.23304639640969782, -275.0757377487332178, -345.3372706006049384 ) ) ;
#341=CARTESIAN_POINT ( 'NONE',  ( -112.9761763116332247, -289.5785814991315874, -283.9848390634267048 ) ) ;
#342=CARTESIAN_POINT ( 'NONE',  ( 21.95725545762149977, -292.5613560969318314, -314.2937286855417938 ) ) ;
#343=CARTESIAN_POINT ( 'NONE',  ( -85.44055784739148862, -276.4180553261052182, -325.9960111145832116 ) ) ;
#344=CARTESIAN_POINT ( 'NONE',  ( -95.72722165873599920, -271.2710829947001230, -224.1827130997946256 ) ) ;
#345=CARTESIAN_POINT ( 'NONE',  ( -22.65836053330757238, -293.5592278193776679, -198.3497090604275854 ) ) ;
#346=CARTESIAN_POINT ( 'NONE',  ( -69.85430415644619018, -285.9805209788416391, -337.9475929042657754 ) ) ;
#347=CARTESIAN_POINT ( 'NONE',  ( -36.30347657727352129, -293.5192792618893236, -346.6737098085878870 ) ) ;
#348=CARTESIAN_POINT ( 'NONE',  ( -72.72470772363107017, -291.1292060606908194, -335.1259478652599455 ) ) ;
#349=CARTESIAN_POINT ( 'NONE',  ( -72.93889733817584897, -289.8270235111069155, -203.2136108133159951 ) ) ;
#350=CARTESIAN_POINT ( 'NONE',  ( 21.65667839415024787, -289.5898385970144204, -314.3659227384940777 ) ) ;
#352=CARTESIAN_POINT ( 'NONE',  ( -84.78198129953274531, -290.5284216945488538, -326.1237722561434111 ) ) ;
#354=CARTESIAN_POINT ( 'NONE',  ( 16.41828331231947047, -289.5142829697366551, -325.0047850796670446 ) ) ;
#355=CARTESIAN_POINT ( 'NONE',  ( -69.24261951150045036, -277.6547478299956424, -202.0774387024998475 ) ) ;
#356=CARTESIAN_POINT ( 'NONE',  ( -93.06138155620693908, -279.6124719458072718, -217.1712879536569858 ) ) ;
#357=CARTESIAN_POINT ( 'NONE',  ( -2.906107825339117934, -282.2763205639810167, -339.2229474479840405 ) ) ;
#358=CARTESIAN_POINT ( 'NONE',  ( 32.85528928337881638, -285.2072911852064863, -243.8063626278319873 ) ) ;
#360=CARTESIAN_POINT ( 'NONE',  ( 16.70922893827216171, -280.4128521477969116, -321.3210328012327182 ) ) ;
#362=CARTESIAN_POINT ( 'NONE',  ( -66.39029194718750659, -283.6716376159805009, -201.2150409871211707 ) ) ;
#363=CARTESIAN_POINT ( 'NONE',  ( 122.1069165698472005, 147.2784710008442062, -260.4370889626021608 ) ) ;
#364=CARTESIAN_POINT ( 'NONE',  ( -97.39534768318327451, -276.3970167199631760, -317.4383648314011452 ) ) ;
#365=CARTESIAN_POINT ( 'NONE',  ( -89.66526190333848945, -284.2554813913510543, -214.2198617431564287 ) ) ;
#366=CARTESIAN_POINT ( 'NONE',  ( -76.65960139014248398, -274.3138574429952996, -208.6626223191690030 ) ) ;
#367=CARTESIAN_POINT ( 'NONE',  ( -110.4121956192968952, -292.0160383064796861, -280.8026003379728195 ) ) ;
#368=CARTESIAN_POINT ( 'NONE',  ( -64.70614803693948147, -275.1270252510786349, -199.0042521874292731 ) ) ;
#369=CARTESIAN_POINT ( 'NONE',  ( 31.13961632253437628, -274.8809954078292321, -245.0155703673037237 ) ) ;
#370=CARTESIAN_POINT ( 'NONE',  ( -31.41970177568762068, -296.9776604953191281, -345.1784422849063390 ) ) ;
#371=CARTESIAN_POINT ( 'NONE',  ( -65.44504524589291350, -289.5761160872477262, -342.1056879275396909 ) ) ;
#372=CARTESIAN_POINT ( 'NONE',  ( 36.45377266294208596, -279.8396616290869474, -286.6547727834441162 ) ) ;
#373=CARTESIAN_POINT ( 'NONE',  ( 20.38009769833850271, -292.6951850229471574, -219.3785238948976826 ) ) ;
#374=CARTESIAN_POINT ( 'NONE',  ( -32.12861129292866735, -291.1782324718648169, -197.2989384837379987 ) ) ;
#375=CARTESIAN_POINT ( 'NONE',  ( -41.85144338877410064, -293.1086862314667201, -345.2764462107752479 ) ) ;
#378=CARTESIAN_POINT ( 'NONE',  ( -81.76149366879960212, -290.9364281575888072, -212.2895999433750660 ) ) ;
#380=CARTESIAN_POINT ( 'NONE',  ( -15.49194037015495340, -287.2693386610928314, -196.7164407258930510 ) ) ;
#381=CARTESIAN_POINT ( 'NONE',  ( -53.35057174420112602, -300.3376638359844719, -200.3683826091709648 ) ) ;
#382=CARTESIAN_POINT ( 'NONE',  ( -5.905052913589146080, -293.7076358184812648, -340.3936634569377588 ) ) ;
#383=CARTESIAN_POINT ( 'NONE',  ( -100.9994486081661194, -285.3040589295532072, -312.8942100776160942 ) ) ;
#384=CARTESIAN_POINT ( 'NONE',  ( -87.69296771485265651, -285.1580413244751639, -217.5051830566009698 ) ) ;
#385=CARTESIAN_POINT ( 'NONE',  ( 27.23484507803531329, -276.5905825887086280, -234.7502008270885199 ) ) ;
#386=CARTESIAN_POINT ( 'NONE',  ( 33.90947907481013601, -291.8606329916426034, -292.6123261580082158 ) ) ;
#387=CARTESIAN_POINT ( 'NONE',  ( 23.78235592887573091, -295.8861003879378586, -312.1859408948212149 ) ) ;
#388=CARTESIAN_POINT ( 'NONE',  ( 34.27735924785553578, -274.5585016382564731, -286.4756392014268158 ) ) ;
#389=ORIENTED_EDGE ( 'NONE', *, *, #16197, .T. ) ;
#391=CARTESIAN_POINT ( 'NONE',  ( 1.755039088397472469, -294.2108378408647127, -336.6724237618244047 ) ) ;
#392=CARTESIAN_POINT ( 'NONE',  ( 36.55663044536660067, -289.5882713313104659, -279.3249863250336489 ) ) ;
#393=CARTESIAN_POINT ( 'NONE',  ( 27.34393682368281375, -296.8617045556625271, -195.3831644147898032 ) ) ;
#394=CARTESIAN_POINT ( 'NONE',  ( -102.0629304562351791, -298.1732284488088567, -229.2192311247754617 ) ) ;
#395=CARTESIAN_POINT ( 'NONE',  ( -25.13295117268265244, -286.8632252611534454, -198.2345166741048388 ) ) ;
#396=CARTESIAN_POINT ( 'NONE',  ( -106.1398451837155505, -277.1705574142181945, -304.5341711825586231 ) ) ;
#397=CARTESIAN_POINT ( 'NONE',  ( -65.55836371735222201, -296.0629673787829006, -341.9094569026487420 ) ) ;
#398=CARTESIAN_POINT ( 'NONE',  ( -65.01824890676496693, -287.5493471980986442, -340.9453832113689487 ) ) ;
#399=CARTESIAN_POINT ( 'NONE',  ( -112.8687659414040212, -297.0724226953441871, -255.4135726666953872 ) ) ;
#401=CARTESIAN_POINT ( 'NONE',  ( -105.7319383130498238, -291.2284431431657481, -244.6273306386740671 ) ) ;
#405=CARTESIAN_POINT ( 'NONE',  ( -110.6395987777366372, -271.3322271728259238, -283.6871839692900039 ) ) ;
#406=CARTESIAN_POINT ( 'NONE',  ( 36.69934693387597235, -288.8392658573746985, -251.9049237673648918 ) ) ;
#407=CARTESIAN_POINT ( 'NONE',  ( -99.86837403722181250, -288.6952119285918457, -220.4570493818173702 ) ) ;
#410=CARTESIAN_POINT ( 'NONE',  ( -110.4501830105272120, -278.2029926013627232, -246.3497191025504947 ) ) ;
#411=CARTESIAN_POINT ( 'NONE',  ( -77.07960880002397630, -285.5857159168178896, -333.8331689869217485 ) ) ;
#412=CARTESIAN_POINT ( 'NONE',  ( -111.3091925084824112, -282.8845413066624701, -289.5811479901594794 ) ) ;
#413=VECTOR ( 'NONE', #28280, 1000.000000000000000 ) ;
#414=CARTESIAN_POINT ( 'NONE',  ( 30.73219615365270485, -286.0310267411410905, -300.6096502203043315 ) ) ;
#415=CARTESIAN_POINT ( 'NONE',  ( 9.776714872701816716, -278.2721951864857601, -329.7590680726313508 ) ) ;
#416=CARTESIAN_POINT ( 'NONE',  ( -110.1599951406477516, -296.9581660565513062, -276.9113938487936366 ) ) ;
#418=CARTESIAN_POINT ( 'NONE',  ( -61.18891464443646555, -294.0530483757174238, -339.9316314393639686 ) ) ;
#419=CARTESIAN_POINT ( 'NONE',  ( -71.19720023784525154, -280.2683243496197179, -201.3167996104560018 ) ) ;
#420=CARTESIAN_POINT ( 'NONE',  ( -95.61175034384609717, -279.1700810579507106, -226.3676360124166536 ) ) ;
#421=CARTESIAN_POINT ( 'NONE',  ( -104.5325035349209770, -278.2870535611997980, -241.5637464807761603 ) ) ;
#422=CARTESIAN_POINT ( 'NONE',  ( -15.87710889929866376, -275.4030008116405384, -196.6801677939435820 ) ) ;
#423=CARTESIAN_POINT ( 'NONE',  ( -82.37591756080814775, -276.5714600047618319, -332.4369729437565866 ) ) ;
#424=CARTESIAN_POINT ( 'NONE',  ( -113.3918672577102740, -270.6791253856088133, -283.7747343605257129 ) ) ;
#425=CARTESIAN_POINT ( 'NONE',  ( -67.97318274279425054, -296.8717553275860723, -340.3633934241867678 ) ) ;
#426=CARTESIAN_POINT ( 'NONE',  ( -69.91165696735023971, -276.1233781216988064, -202.8022627189028810 ) ) ;
#428=CARTESIAN_POINT ( 'NONE',  ( 7.103459944063120091, -287.7531359562102580, -211.9972993146364217 ) ) ;
#429=CARTESIAN_POINT ( 'NONE',  ( -69.38620004629432003, -287.3964490037180326, -201.4475639410760834 ) ) ;
#430=CARTESIAN_POINT ( 'NONE',  ( 35.06017669879758358, -287.0348881638780085, -280.5447993308172272 ) ) ;
#431=CARTESIAN_POINT ( 'NONE',  ( 24.20210434625752782, -281.6748354658932953, -316.5334802164283019 ) ) ;
#432=CARTESIAN_POINT ( 'NONE',  ( -110.7597969522451393, -277.0562332315128629, -262.3744125087495718 ) ) ;
#433=CARTESIAN_POINT ( 'NONE',  ( -98.53737060242386292, -285.8362405327920328, -312.4739421121791452 ) ) ;
#434=CARTESIAN_POINT ( 'NONE',  ( -98.55886781794781371, -277.5975963507496544, -229.2441326131148003 ) ) ;
#435=CARTESIAN_POINT ( 'NONE',  ( -18.87697925039016056, -278.1245800897174263, -341.4968864787559824 ) ) ;
#436=CARTESIAN_POINT ( 'NONE',  ( 7.363625341111400324, -275.1731506385693251, -212.5733829849779397 ) ) ;
#437=CARTESIAN_POINT ( 'NONE',  ( -43.16748347093800930, -287.9191015667062175, -346.7421952665334857 ) ) ;
#439=CARTESIAN_POINT ( 'NONE',  ( -34.47473844410745158, -283.8198020982060257, -347.1461383420058269 ) ) ;
#441=CARTESIAN_POINT ( 'NONE',  ( 35.55280058431892343, -282.3566568378734019, -295.1421408184978645 ) ) ;
#445=CARTESIAN_POINT ( 'NONE',  ( 11.63567796159732204, -290.2411052206740578, -328.1670165858570272 ) ) ;
#448=CARTESIAN_POINT ( 'NONE',  ( -101.2626605397846049, -289.7943000246049223, -228.2255153181214098 ) ) ;
#449=CARTESIAN_POINT ( 'NONE',  ( 94.78702171985756308, -298.9449283184634965, -197.2183506070807653 ) ) ;
#450=CARTESIAN_POINT ( 'NONE',  ( -11.09980241159285619, -294.0676480132073607, -342.6995274442535901 ) ) ;
#451=CARTESIAN_POINT ( 'NONE',  ( 35.64438321566538548, -286.1663195541688651, -280.6380762210182525 ) ) ;
#452=CARTESIAN_POINT ( 'NONE',  ( 36.05237603647821487, -288.7659386966579405, -271.0245089406109855 ) ) ;
#453=CARTESIAN_POINT ( 'NONE',  ( 21.27581636871892101, -289.4090924074130839, -223.5744983911110353 ) ) ;
#454=CARTESIAN_POINT ( 'NONE',  ( 37.35780284020656694, -289.6384337990135691, -277.0681965735167296 ) ) ;
#455=CARTESIAN_POINT ( 'NONE',  ( -102.9959811661897078, -289.0380696731132275, -233.7613392213682744 ) ) ;
#456=CARTESIAN_POINT ( 'NONE',  ( -41.38985635712994338, -294.0013616208397025, -195.4577283638537892 ) ) ;
#457=CARTESIAN_POINT ( 'NONE',  ( -108.9475998404428339, -285.2906192478001230, -285.7830426642873931 ) ) ;
#458=CARTESIAN_POINT ( 'NONE',  ( -44.74250737014229884, -293.9589824279485128, -195.5080083575545302 ) ) ;
#461=CARTESIAN_POINT ( 'NONE',  ( -69.45425524740572598, -275.6116147604159892, -202.1767048456104305 ) ) ;
#462=CARTESIAN_POINT ( 'NONE',  ( 34.22529250880975127, -280.5486076104474478, -255.1103591393745091 ) ) ;
#463=CARTESIAN_POINT ( 'NONE',  ( -5.198279291450013773, -280.6290538813578337, -338.1380734097782010 ) ) ;
#464=CARTESIAN_POINT ( 'NONE',  ( -107.0242423197752260, -295.3340369974355895, -302.7417006471805507 ) ) ;
#465=CARTESIAN_POINT ( 'NONE',  ( 26.15657362997979973, -273.2749777785776359, -232.2362400515366687 ) ) ;
#466=CARTESIAN_POINT ( 'NONE',  ( -67.40623058219914299, -275.5294293008589648, -338.4598566561462576 ) ) ;
#467=CARTESIAN_POINT ( 'NONE',  ( -70.70629809753577888, -298.9177607521856430, -204.8639294649306635 ) ) ;
#468=AXIS2_PLACEMENT_3D ( 'NONE', #23626, #88479, #15587 ) ;
#469=CARTESIAN_POINT ( 'NONE',  ( -12.79472286548296189, -296.1521451354898318, -339.7893085137351363 ) ) ;
#472=CARTESIAN_POINT ( 'NONE',  ( -93.19907288353067543, -296.6847407908389300, -317.6304496190813325 ) ) ;
#473=DIRECTION ( 'NONE',  ( -0.8510748438184358999, -0.5250018354872690862, -0.006684530980050039546 ) ) ;
#475=CARTESIAN_POINT ( 'NONE',  ( -62.62531095629989153, -283.7448301468398881, -199.3741767513798777 ) ) ;
#476=CARTESIAN_POINT ( 'NONE',  ( -108.7791315055169292, -296.7511089224530565, -255.2779189747055852 ) ) ;
#478=CARTESIAN_POINT ( 'NONE',  ( -104.0404571924912176, -285.0535134706426561, -231.7807334197285059 ) ) ;
#479=CARTESIAN_POINT ( 'NONE',  ( 38.08672107127473794, -287.4111732831478889, -285.7330914080269508 ) ) ;
#480=CARTESIAN_POINT ( 'NONE',  ( -27.84916182087626524, -290.1726618128096788, -196.0802578231074733 ) ) ;
#482=CARTESIAN_POINT ( 'NONE',  ( -96.68618260603486192, -278.4065655959097398, -221.5309156116981342 ) ) ;
#483=CARTESIAN_POINT ( 'NONE',  ( -110.4683760289727132, -275.8380690714489560, -287.0191576251351080 ) ) ;
#486=CARTESIAN_POINT ( 'NONE',  ( 15.32504751799938170, -285.6119886687430949, -219.2402396929666111 ) ) ;
#487=CARTESIAN_POINT ( 'NONE',  ( -110.1331340237950371, -289.7794927530383688, -246.0517078306988310 ) ) ;
#489=FACE_OUTER_BOUND ( 'NONE', #65073, .T. ) ;
#490=CARTESIAN_POINT ( 'NONE',  ( -94.54989721759596932, -297.4992510617885841, -317.0035278207499232 ) ) ;
#491=CARTESIAN_POINT ( 'NONE',  ( -2.673819891810099048, -281.9266918661726891, -202.2528603128815234 ) ) ;
#492=CARTESIAN_POINT ( 'NONE',  ( -112.0260394306532987, -294.4391519622371902, -280.7769840364173888 ) ) ;
#493=CARTESIAN_POINT ( 'NONE',  ( 33.66971584016666696, -281.4439457894184216, -287.4280102006902666 ) ) ;
#494=CARTESIAN_POINT ( 'NONE',  ( 28.10704333086922801, -294.2504591929128992, -311.0255889924686130 ) ) ;
#496=ADVANCED_FACE ( 'NONE', ( #85859 ), #33336, .T. ) ;
#497=CARTESIAN_POINT ( 'NONE',  ( -67.88206223731559419, -281.6514772224624039, -201.8468337845070266 ) ) ;
#498=CARTESIAN_POINT ( 'NONE',  ( -106.2125426076041634, -295.2784407768329515, -295.4144270085473636 ) ) ;
#502=CARTESIAN_POINT ( 'NONE',  ( -95.55218877742616712, -285.8860174903883831, -317.1081560315652155 ) ) ;
#504=CARTESIAN_POINT ( 'NONE',  ( -110.4542110544635705, -282.2666405000204009, -253.6410175316879361 ) ) ;
#505=CARTESIAN_POINT ( 'NONE',  ( -1.368022843707428438, -273.7141166933243994, -202.4637442224215818 ) ) ;
#506=CARTESIAN_POINT ( 'NONE',  ( -109.9726748286922628, -290.4821773897211301, -263.0302572872621454 ) ) ;
#507=CARTESIAN_POINT ( 'NONE',  ( 25.71966169681331849, -282.5511572894125152, -232.1312805657929346 ) ) ;
#508=CARTESIAN_POINT ( 'NONE',  ( -96.93934988317018053, -274.7561529871699690, -226.7496344372156614 ) ) ;
#510=CARTESIAN_POINT ( 'NONE',  ( 33.84745103067382388, -283.4999324435455037, -297.5373055610141364 ) ) ;
#511=CARTESIAN_POINT ( 'NONE',  ( 22.12468463488144010, -280.9459354239748450, -313.4044813569679491 ) ) ;
#512=CARTESIAN_POINT ( 'NONE',  ( -111.1035872555647188, -280.7265676192138812, -256.7896531230614983 ) ) ;
#513=CARTESIAN_POINT ( 'NONE',  ( -90.16440307809195076, -273.4969061714966756, -214.2636476280938780 ) ) ;
#514=CARTESIAN_POINT ( 'NONE',  ( 2.419818390556676135, -274.4029431552878009, -204.4215877325289057 ) ) ;
#515=CARTESIAN_POINT ( 'NONE',  ( 35.04236977698502642, -295.2468850698101619, -252.9326020219452857 ) ) ;
#517=CARTESIAN_POINT ( 'NONE',  ( 16.66419048074589782, -292.4339046538751177, -323.5739229754051394 ) ) ;
#518=CARTESIAN_POINT ( 'NONE',  ( 5.217678648793666163, -274.1526882925118684, -210.9126626711573067 ) ) ;
#519=CARTESIAN_POINT ( 'NONE',  ( -76.82721684469869672, -293.0540813855774900, -205.0039100937321734 ) ) ;
#520=CARTESIAN_POINT ( 'NONE',  ( -110.4683760289727132, -275.2662352645559167, -253.7030783399848985 ) ) ;
#521=CARTESIAN_POINT ( 'NONE',  ( -33.57432131573970224, -293.3036558292391760, -193.8508861434929997 ) ) ;
#522=CARTESIAN_POINT ( 'NONE',  ( 32.19804620522597105, -289.9147606758254483, -298.1461082847454236 ) ) ;
#523=CARTESIAN_POINT ( 'NONE',  ( -102.1838148814982645, -276.0511314017147129, -307.8220257815003720 ) ) ;
#524=CARTESIAN_POINT ( 'NONE',  ( -73.52089337593383789, -279.4562368179799705, -335.4325269178318649 ) ) ;
#525=CARTESIAN_POINT ( 'NONE',  ( -34.26569199195837712, -293.0930187872357351, -344.7375414908350422 ) ) ;
#526=CARTESIAN_POINT ( 'NONE',  ( 18.23768133693696214, -282.6996858500997973, -218.8709457477553144 ) ) ;
#528=CARTESIAN_POINT ( 'NONE',  ( -66.57193366333181928, -283.1125662302549699, -337.2901694264401158 ) ) ;
#529=CARTESIAN_POINT ( 'NONE',  ( -79.75134091025527994, -280.5733721980102473, -206.3997167747376125 ) ) ;
#531=CARTESIAN_POINT ( 'NONE',  ( 35.22795202031545614, -280.6595075427375150, -295.0545065737637174 ) ) ;
#532=CARTESIAN_POINT ( 'NONE',  ( -59.58534422498445338, -278.2746395945201812, -343.8324764135672922 ) ) ;
#534=CARTESIAN_POINT ( 'NONE',  ( -6.833954875992621858, -278.1790821057300604, -340.3179759246217486 ) ) ;
#535=CARTESIAN_POINT ( 'NONE',  ( -102.0455923789670294, -281.4805209788416960, -239.2376011013261916 ) ) ;
#538=CARTESIAN_POINT ( 'NONE',  ( -94.27891396533529189, -299.2288517735989899, -221.5237939030694179 ) ) ;
#540=CARTESIAN_POINT ( 'NONE',  ( -51.61964741925273614, -275.2557921787226292, -343.6276657439970563 ) ) ;
#541=CARTESIAN_POINT ( 'NONE',  ( -39.20955032075062263, -293.7891813239779140, -194.3845451917290461 ) ) ;
#542=CARTESIAN_POINT ( 'NONE',  ( 29.58004740640543417, -293.2959480609137017, -299.7783302023191254 ) ) ;
#543=CARTESIAN_POINT ( 'NONE',  ( 32.65864715560118725, -286.6498733850967255, -238.3035732600245922 ) ) ;
#545=CARTESIAN_POINT ( 'NONE',  ( -22.23194966639039194, -293.4369986843219635, -345.2630654359047639 ) ) ;
#546=CARTESIAN_POINT ( 'NONE',  ( -108.5382654350417795, -282.6975571727014653, -289.8379683928316126 ) ) ;
#547=CARTESIAN_POINT ( 'NONE',  ( -64.24683902220084519, -291.2672496188426408, -339.6042094105640672 ) ) ;
#548=CARTESIAN_POINT ( 'NONE',  ( -108.0627017584748870, -282.7599712521561628, -291.1245075829212965 ) ) ;
#549=CARTESIAN_POINT ( 'NONE',  ( 25.99246253114274552, -283.3771681065013013, -307.7447886190831241 ) ) ;
#550=CARTESIAN_POINT ( 'NONE',  ( -45.98732877144905018, -290.1003550732238523, -346.6903779564393062 ) ) ;
#552=CARTESIAN_POINT ( 'NONE',  ( -27.55633526468844252, -280.6720254424021164, -197.9066035369142469 ) ) ;
#553=CARTESIAN_POINT ( 'NONE',  ( -33.47033252515218749, -293.7993959282042056, -346.8792103833187639 ) ) ;
#554=CARTESIAN_POINT ( 'NONE',  ( -37.49099266878829440, -289.8567683557566852, -347.2125418609350049 ) ) ;
#555=CARTESIAN_POINT ( 'NONE',  ( 12.38083513092553289, -288.8732566723153354, -329.0739478451774289 ) ) ;
#556=CARTESIAN_POINT ( 'NONE',  ( -8.256898078943684993, -286.6106324874740494, -203.4053542703483117 ) ) ;
#559=CARTESIAN_POINT ( 'NONE',  ( 12.59971999844131396, -296.2254926977316813, -327.4057811323250462 ) ) ;
#560=CIRCLE ( 'NONE', #36843, 1.897123461337413275 ) ;
#561=CARTESIAN_POINT ( 'NONE',  ( -113.6276753064661165, -295.3183646335438652, -263.8953553310242910 ) ) ;
#562=CARTESIAN_POINT ( 'NONE',  ( -109.7264424368263178, -277.4645562237244008, -281.4902477421676394 ) ) ;
#563=CARTESIAN_POINT ( 'NONE',  ( 98.96984324953363910, -299.0653406705604880, -193.4775484312997662 ) ) ;
#564=CARTESIAN_POINT ( 'NONE',  ( -12.79537854053787704, -293.2072255931282143, -339.9000241336492536 ) ) ;
#565=CARTESIAN_POINT ( 'NONE',  ( 33.01822646521787874, -277.0097735718116496, -247.2300213676486464 ) ) ;
#566=CARTESIAN_POINT ( 'NONE',  ( -35.08692667047458258, -296.3206129209522146, -196.3484649373850175 ) ) ;
#567=CARTESIAN_POINT ( 'NONE',  ( 36.10541241948924807, -294.7622949125877767, -270.7467767446918856 ) ) ;
#568=CARTESIAN_POINT ( 'NONE',  ( 26.06689073608121276, -295.1344300300592636, -307.1521043461206659 ) ) ;
#571=CARTESIAN_POINT ( 'NONE',  ( -97.60692826702394598, -295.1643581662601719, -225.4160354886601851 ) ) ;
#572=CARTESIAN_POINT ( 'NONE',  ( -9.165054654810878887, -299.0476583445857841, -193.4600241329953008 ) ) ;
#574=CARTESIAN_POINT ( 'NONE',  ( -68.84837883859820806, -290.4181530666822368, -336.4726725368212783 ) ) ;
#575=CARTESIAN_POINT ( 'NONE',  ( -28.88931899185833885, -295.2754706862511966, -342.9424488748248905 ) ) ;
#576=CARTESIAN_POINT ( 'NONE',  ( -93.95798993011017330, -279.8443368349776392, -320.0904104946291682 ) ) ;
#577=CARTESIAN_POINT ( 'NONE',  ( -113.2789115823150041, -277.1143977978192652, -280.1000033892999568 ) ) ;
#579=CARTESIAN_POINT ( 'NONE',  ( 19.70231359237515179, -281.6026258314327038, -322.0073482961647642 ) ) ;
#580=CARTESIAN_POINT ( 'NONE',  ( 36.49033549754070549, -274.6286845839015314, -248.6774485503754875 ) ) ;
#581=CARTESIAN_POINT ( 'NONE',  ( -56.71680268613243925, -281.3837387631637625, -342.2354499514945587 ) ) ;
#582=CARTESIAN_POINT ( 'NONE',  ( -45.17069689039524860, -278.3545798726502767, -194.5119291036368736 ) ) ;
#583=CARTESIAN_POINT ( 'NONE',  ( -22.89302449604697998, -278.2363000005352660, -196.5432261782136436 ) ) ;
#585=CARTESIAN_POINT ( 'NONE',  ( -71.88205993780856318, -296.2703597272860065, -205.4761310522087570 ) ) ;
#586=CARTESIAN_POINT ( 'NONE',  ( 37.31721839381581418, -277.6507211666369130, -278.0251792108447830 ) ) ;
#588=CARTESIAN_POINT ( 'NONE',  ( -22.49268826115504893, -290.2613106025819434, -196.4302554823797493 ) ) ;
#589=CARTESIAN_POINT ( 'NONE',  ( -107.7313703303886285, -290.1523481562727511, -301.7059457455363258 ) ) ;
#591=CARTESIAN_POINT ( 'NONE',  ( -60.33512634693056498, -275.7550055312672157, -198.7433316086200819 ) ) ;
#592=CARTESIAN_POINT ( 'NONE',  ( -94.41974712616571708, -271.2258015954081429, -221.6884789025067164 ) ) ;
#593=CARTESIAN_POINT ( 'NONE',  ( -110.7686810774425936, -284.0362970395182174, -247.5406166420813747 ) ) ;
#595=CARTESIAN_POINT ( 'NONE',  ( -42.85221553818946205, -283.9824678662702127, -195.5510574499011227 ) ) ;
#597=CARTESIAN_POINT ( 'NONE',  ( -34.82839873673886899, -290.8793472931504311, -197.0070872693103183 ) ) ;
#598=CARTESIAN_POINT ( 'NONE',  ( -109.2187920824703014, -282.9326966191597421, -251.7990832069660883 ) ) ;
#601=CARTESIAN_POINT ( 'NONE',  ( 37.19157926738635211, -291.6650951418104114, -279.1700606143812706 ) ) ;
#602=CARTESIAN_POINT ( 'NONE',  ( -55.55561266974274304, -281.7623218828950939, -344.4621378191625354 ) ) ;
#603=CARTESIAN_POINT ( 'NONE',  ( -108.5873101429798737, -279.9007832254608843, -289.6095846808224223 ) ) ;
#604=CARTESIAN_POINT ( 'NONE',  ( -100.6768922541744047, -286.3294367639458073, -227.1783866267950032 ) ) ;
#605=CARTESIAN_POINT ( 'NONE',  ( -69.98243004323033745, -285.6098162693991753, -205.0510579513368725 ) ) ;
#606=CARTESIAN_POINT ( 'NONE',  ( -26.92027407178215270, -278.3423156410380557, -343.2086903171750123 ) ) ;
#607=CARTESIAN_POINT ( 'NONE',  ( -110.3286395538065392, -279.2794286552243079, -276.1017110174043978 ) ) ;
#609=CARTESIAN_POINT ( 'NONE',  ( -72.69342520872417879, -287.5845644191949191, -204.1578700096011403 ) ) ;
#612=CARTESIAN_POINT ( 'NONE',  ( -36.27657800195181892, -294.8725021804859239, -347.3668546410453359 ) ) ;
#613=CARTESIAN_POINT ( 'NONE',  ( 35.62372540500069107, -289.7358906677945356, -286.1657956460347805 ) ) ;
#615=CARTESIAN_POINT ( 'NONE',  ( 25.18497378105907814, -277.4090924074130839, -220.4570493818173702 ) ) ;
#616=CARTESIAN_POINT ( 'NONE',  ( 36.65006893773713159, -291.7218174702185820, -252.1496235759580600 ) ) ;
#618=CARTESIAN_POINT ( 'NONE',  ( -16.99888552950729448, -287.8396185546561128, -199.4778519094652438 ) ) ;
#619=CARTESIAN_POINT ( 'NONE',  ( -108.5999294765276062, -280.5736674880837995, -250.3081247049989599 ) ) ;
#620=CARTESIAN_POINT ( 'NONE',  ( 5.244095234645274495, -289.9134760916920186, -333.8044495868525701 ) ) ;
#621=CARTESIAN_POINT ( 'NONE',  ( -66.05854980302595436, -285.4280788811326488, -339.6595958286496852 ) ) ;
#622=CARTESIAN_POINT ( 'NONE',  ( -102.0958390393031152, -278.1710745719942111, -312.1225588290878363 ) ) ;
#623=ORIENTED_EDGE ( 'NONE', *, *, #12372, .T. ) ;
#624=CARTESIAN_POINT ( 'NONE',  ( 38.16695403606040315, -291.6674930577466398, -273.1463184486848377 ) ) ;
#625=CARTESIAN_POINT ( 'NONE',  ( 38.14512944601662525, -281.5754459229366375, -285.5511991337033351 ) ) ;
#627=CARTESIAN_POINT ( 'NONE',  ( -91.10728457839564953, -275.1385753027915371, -219.1553335681576300 ) ) ;
#630=CARTESIAN_POINT ( 'NONE',  ( -4.771743288812468897, -297.1233781216987495, -337.9199732462171255 ) ) ;
#631=CARTESIAN_POINT ( 'NONE',  ( -1.755944882127600470, -272.7569627845279001, -203.2222466845226450 ) ) ;
#633=CARTESIAN_POINT ( 'NONE',  ( -93.13313667296279164, -278.7298411586599514, -223.1687471948053485 ) ) ;
#635=CARTESIAN_POINT ( 'NONE',  ( 22.34134370700455108, -277.4043121424948595, -318.4021071408388366 ) ) ;
#636=CARTESIAN_POINT ( 'NONE',  ( -47.37087138965788569, -299.3476306537725691, -197.4068819803149779 ) ) ;
#637=CARTESIAN_POINT ( 'NONE',  ( -30.24860219207629086, -282.0232362878585946, -346.7974194006311563 ) ) ;
#638=CARTESIAN_POINT ( 'NONE',  ( -82.36296692948907605, -293.1885541418192247, -211.5505299430354853 ) ) ;
#639=CARTESIAN_POINT ( 'NONE',  ( 97.63982572653510772, -301.2333003928553694, -194.0202035235065523 ) ) ;
#640=CARTESIAN_POINT ( 'NONE',  ( -29.12807470841969959, -299.3579053438171513, -193.7565484485259617 ) ) ;
#641=CARTESIAN_POINT ( 'NONE',  ( 13.62160783359252392, -296.3369496282019782, -325.2296967268541721 ) ) ;
#642=CARTESIAN_POINT ( 'NONE',  ( -77.12276404418378206, -281.5860396746064112, -333.8061287737435805 ) ) ;
#643=CARTESIAN_POINT ( 'NONE',  ( -49.11044639364758524, -271.9217030055709188, -196.5975770573392083 ) ) ;
#644=CARTESIAN_POINT ( 'NONE',  ( 4.720918495268251469, -288.2095907686901910, -206.7595012800831853 ) ) ;
#646=CARTESIAN_POINT ( 'NONE',  ( -0.8494590164562774159, -287.4760563537427061, -334.0005347574279995 ) ) ;
#647=CARTESIAN_POINT ( 'NONE',  ( 204.7385211771276090, 294.9049021488058315, -68.64726399651360111 ) ) ;
#649=CARTESIAN_POINT ( 'NONE',  ( -82.51898930543246991, -288.2306517282796108, -331.9859411788225430 ) ) ;
#650=CARTESIAN_POINT ( 'NONE',  ( -10.72034586036382287, -288.3620045295733689, -338.4108699226561043 ) ) ;
#652=CARTESIAN_POINT ( 'NONE',  ( -60.43001306444523379, -286.8393884576937580, -197.1728528206301689 ) ) ;
#653=CARTESIAN_POINT ( 'NONE',  ( -36.46166220244045064, -277.3741405195800098, -343.3894296830907820 ) ) ;
#654=CARTESIAN_POINT ( 'NONE',  ( 31.91276623249945388, -292.0471199576754771, -237.2935922219214149 ) ) ;
#655=CARTESIAN_POINT ( 'NONE',  ( -114.1060177499678190, -285.1364680378219418, -275.7189543159105369 ) ) ;
#656=CARTESIAN_POINT ( 'NONE',  ( 27.25401748960190673, -282.5344009542761228, -229.6406980113972054 ) ) ;
#657=CARTESIAN_POINT ( 'NONE',  ( -30.21262458242523508, -283.2975638927446767, -347.0091484423581392 ) ) ;
#658=CARTESIAN_POINT ( 'NONE',  ( 23.69787251492912006, -281.3288461764117869, -230.1917899458019576 ) ) ;
#659=CARTESIAN_POINT ( 'NONE',  ( 45.39964763510799628, 12.39790288765882842, -332.1295406407559199 ) ) ;
#660=CARTESIAN_POINT ( 'NONE',  ( -111.9891808443444461, -280.6201449729597357, -265.0902502256173534 ) ) ;
#661=CARTESIAN_POINT ( 'NONE',  ( 184.0236931359747246, 263.5994396450613522, -152.8319179813719870 ) ) ;
#662=CARTESIAN_POINT ( 'NONE',  ( 166.1890715538564791, 230.9239408293323095, -190.2239395719806510 ) ) ;
#663=CARTESIAN_POINT ( 'NONE',  ( -78.93849876691669465, -272.6728204782807552, -210.1139715849992058 ) ) ;
#664=CARTESIAN_POINT ( 'NONE',  ( 0.5047639842331865800, -294.0694645151006625, -337.3626420394939487 ) ) ;
#665=CARTESIAN_POINT ( 'NONE',  ( -97.29061877149726456, -247.0397287528579113, -331.5487825117278362 ) ) ;
#666=CARTESIAN_POINT ( 'NONE',  ( -13.20211036784315972, -273.0441534182189685, -197.7623681437754328 ) ) ;
#667=CARTESIAN_POINT ( 'NONE',  ( -40.59542752110353803, -299.8712516084596587, -196.1844929354027443 ) ) ;
#668=CARTESIAN_POINT ( 'NONE',  ( 35.01011000808389184, -289.0363855024123154, -283.2630189616197640 ) ) ;
#670=CARTESIAN_POINT ( 'NONE',  ( -47.58826728983434862, -296.1206370813446824, -346.4388944609972896 ) ) ;
#671=CARTESIAN_POINT ( 'NONE',  ( 2.475306229651003775, -287.0942543838424399, -209.1026945105221841 ) ) ;
#672=CARTESIAN_POINT ( 'NONE',  ( -91.93931476158491023, -272.2152748747753321, -216.5039644581051164 ) ) ;
#673=CARTESIAN_POINT ( 'NONE',  ( 39.07760704016652653, -294.4615816861127655, -278.8668147344420731 ) ) ;
#674=CARTESIAN_POINT ( 'NONE',  ( 30.85070177834801441, -294.5045078308516509, -305.9886807015176942 ) ) ;
#675=CARTESIAN_POINT ( 'NONE',  ( -92.55788908050703867, -291.3992417568560427, -222.6099663514978602 ) ) ;
#677=CARTESIAN_POINT ( 'NONE',  ( -10.87534909323254162, -276.3145722300414491, -199.5322585787767764 ) ) ;
#678=CARTESIAN_POINT ( 'NONE',  ( 30.18575029894034856, -274.8182300232326156, -306.6400819815780210 ) ) ;
#681=CARTESIAN_POINT ( 'NONE',  ( -98.75809043947947430, -277.4419339083197542, -316.7244509340659420 ) ) ;
#682=CARTESIAN_POINT ( 'NONE',  ( 34.01050524860151825, -274.1982273214497923, -289.2106061636620780 ) ) ;
#683=CARTESIAN_POINT ( 'NONE',  ( -83.39540030172024387, -274.4831417728582323, -213.3235621710938972 ) ) ;
#685=CARTESIAN_POINT ( 'NONE',  ( 15.60864973082017393, -275.7652360154463622, -219.6945515725571170 ) ) ;
#686=CARTESIAN_POINT ( 'NONE',  ( -69.72061775601729039, -275.3918994113864755, -201.6040406954463435 ) ) ;
#687=CARTESIAN_POINT ( 'NONE',  ( 37.98731941993962380, -273.5468729298579547, -268.3747610727709798 ) ) ;
#688=CARTESIAN_POINT ( 'NONE',  ( -73.34539347806307319, -296.1946930322869207, -333.9820794140245539 ) ) ;
#689=CARTESIAN_POINT ( 'NONE',  ( 32.90389529345434738, -292.4151633868495423, -292.2912625614695230 ) ) ;
#691=CARTESIAN_POINT ( 'NONE',  ( -73.74206659050952339, -280.0745212260765697, -202.5631407710726535 ) ) ;
#692=CARTESIAN_POINT ( 'NONE',  ( 0.6106540497750301277, -274.7402250509520627, -208.0023269674989308 ) ) ;
#694=CARTESIAN_POINT ( 'NONE',  ( -113.6585905315610887, -283.3136399340182834, -264.2707121798462140 ) ) ;
#695=CARTESIAN_POINT ( 'NONE',  ( -92.33048596441228995, -297.8364558181106077, -321.6271343944029013 ) ) ;
#697=CARTESIAN_POINT ( 'NONE',  ( -44.02897957833364018, -285.1626039587596892, -197.5059052623096534 ) ) ;
#699=CARTESIAN_POINT ( 'NONE',  ( -97.21239272151814248, -277.3926882713108171, -226.8470491839136400 ) ) ;
#700=CARTESIAN_POINT ( 'NONE',  ( -29.66990048082298514, -275.5279792476659395, -343.6006735400557659 ) ) ;
#701=CARTESIAN_POINT ( 'NONE',  ( -82.90715564395567583, -285.6751684639340283, -329.9973929718272529 ) ) ;
#702=CARTESIAN_POINT ( 'NONE',  ( 31.48537372293037961, -276.4191044763052787, -244.8667184141149846 ) ) ;
#704=CARTESIAN_POINT ( 'NONE',  ( 34.44041461593528908, -274.2798963078302563, -296.0854221206491843 ) ) ;
#705=CARTESIAN_POINT ( 'NONE',  ( -45.10985561628647389, -281.9542883495410024, -195.5451983406714476 ) ) ;
#707=CARTESIAN_POINT ( 'NONE',  ( 23.00713597926944942, -290.0892507473819819, -315.8290427371612736 ) ) ;
#708=CARTESIAN_POINT ( 'NONE',  ( 36.16907749350749413, -291.7437606598707589, -285.2963673797056003 ) ) ;
#710=CARTESIAN_POINT ( 'NONE',  ( -93.27831109108397811, -271.9106773320791035, -222.6726400747448054 ) ) ;
#711=CARTESIAN_POINT ( 'NONE',  ( -94.37384017523662294, -289.3549625681253588, -222.8207545989157836 ) ) ;
#712=CARTESIAN_POINT ( 'NONE',  ( 202.1133578493929974, 280.9843981858382449, -111.1516734208197050 ) ) ;
#713=CARTESIAN_POINT ( 'NONE',  ( -71.35234327475265559, -295.6029625508436425, -203.5016567919726356 ) ) ;
#714=CARTESIAN_POINT ( 'NONE',  ( -93.09953196885054183, -288.3145404164422985, -322.5311680223112489 ) ) ;
#715=CARTESIAN_POINT ( 'NONE',  ( -13.24915408362107350, -284.3342105798197395, -340.1719614645312504 ) ) ;
#716=CARTESIAN_POINT ( 'NONE',  ( -112.1435345831089876, -282.6189540547150045, -284.0168456740346414 ) ) ;
#717=CARTESIAN_POINT ( 'NONE',  ( -68.01354514851423971, -284.8882368152389404, -337.2536649652591336 ) ) ;
#718=CARTESIAN_POINT ( 'NONE',  ( -108.1875804585888972, -285.5955144221215960, -252.1001495632447700 ) ) ;
#719=CARTESIAN_POINT ( 'NONE',  ( -41.64096488500164384, -291.0859193018515612, -345.6065183928104716 ) ) ;
#720=CARTESIAN_POINT ( 'NONE',  ( -29.84516578740547033, -274.4778797707422200, -193.7481539074419175 ) ) ;
#721=CARTESIAN_POINT ( 'NONE',  ( -40.30719237505373087, -287.1689770165053233, -345.8757432178310296 ) ) ;
#722=CARTESIAN_POINT ( 'NONE',  ( 20.82025024435684912, -276.2342150227256639, -320.8408352078911321 ) ) ;
#723=CARTESIAN_POINT ( 'NONE',  ( 37.06597823717751083, -295.6087467872084176, -276.3062168818707391 ) ) ;
#725=CARTESIAN_POINT ( 'NONE',  ( -114.2704648735229114, -293.0519495502703080, -270.3937649182068981 ) ) ;
#726=CARTESIAN_POINT ( 'NONE',  ( -42.98740052095085673, -281.8095809704739168, -343.6875247501199055 ) ) ;
#727=CARTESIAN_POINT ( 'NONE',  ( -98.97715580903263799, -275.9694145354928878, -313.3855183923923278 ) ) ;
#728=CARTESIAN_POINT ( 'NONE',  ( -100.6226321081433781, -271.6000071654493695, -227.6263586771150074 ) ) ;
#729=CARTESIAN_POINT ( 'NONE',  ( -1.427376833368756426, -275.9114168707258159, -334.0898501826283677 ) ) ;
#730=CARTESIAN_POINT ( 'NONE',  ( -4.541713650276184566, -294.0124598401033609, -204.3556340102542777 ) ) ;
#731=CARTESIAN_POINT ( 'NONE',  ( 34.17699636152847376, -294.2853670901897658, -254.5397820205500068 ) ) ;
#732=CARTESIAN_POINT ( 'NONE',  ( -98.96298881946114534, -286.8735947792195589, -229.3636693604602783 ) ) ;
#734=CARTESIAN_POINT ( 'NONE',  ( 20.84983128615508363, -294.3043723182107101, -220.8199075194258683 ) ) ;
#735=CARTESIAN_POINT ( 'NONE',  ( 36.93909827691977199, -294.6366481941321922, -252.0400573451966295 ) ) ;
#736=CARTESIAN_POINT ( 'NONE',  ( -104.9627000912016257, -296.0170608139034698, -297.8638518189455340 ) ) ;
#737=CARTESIAN_POINT ( 'NONE',  ( -85.96274351581530482, -291.7255569088807192, -327.5347675078998577 ) ) ;
#738=CARTESIAN_POINT ( 'NONE',  ( -16.13979987481713607, -282.9521913927768537, -344.4399102074102643 ) ) ;
#739=CARTESIAN_POINT ( 'NONE',  ( -95.07089606665093129, -271.3642186167389809, -221.2733869658146659 ) ) ;
#740=CARTESIAN_POINT ( 'NONE',  ( 14.24845483363844245, -286.5864904423447683, -213.1279171234522209 ) ) ;
#741=CARTESIAN_POINT ( 'NONE',  ( -90.23390132372703931, -279.7841386887515114, -323.1057526331036911 ) ) ;
#743=CARTESIAN_POINT ( 'NONE',  ( -110.0031653911141376, -283.4830689082544950, -259.9956961012273950 ) ) ;
#744=CARTESIAN_POINT ( 'NONE',  ( 13.23568978385866401, -286.3453118881884052, -325.8113266033782907 ) ) ;
#745=CARTESIAN_POINT ( 'NONE',  ( -40.92587324162294493, -278.1471230759572677, -194.6681552588967747 ) ) ;
#746=CARTESIAN_POINT ( 'NONE',  ( -111.6667267435858832, -264.5695759149226092, -294.5014218916285245 ) ) ;
#747=CARTESIAN_POINT ( 'NONE',  ( -72.39803528208439332, -285.0825930300327400, -206.2450818814191393 ) ) ;
#748=CARTESIAN_POINT ( 'NONE',  ( 27.50698835981510015, -282.2194054974996789, -229.4860579828455514 ) ) ;
#749=CARTESIAN_POINT ( 'NONE',  ( -34.68699798678275670, -288.0783086793965708, -347.0799081848566061 ) ) ;
#750=CARTESIAN_POINT ( 'NONE',  ( -34.30239203478355847, -278.6146582274110983, -346.5004837745580062 ) ) ;
#751=CARTESIAN_POINT ( 'NONE',  ( -1.682637469674603148, -277.9047561968292257, -338.0495920695061614 ) ) ;
#752=CARTESIAN_POINT ( 'NONE',  ( -59.73161367698386925, -279.5873447164300387, -200.8262205653199999 ) ) ;
#753=CARTESIAN_POINT ( 'NONE',  ( -29.84929053798609999, -276.1273659102687930, -196.0932877960297844 ) ) ;
#754=CARTESIAN_POINT ( 'NONE',  ( 30.90234519700421600, -294.0122398859246005, -306.0227258777134125 ) ) ;
#755=CARTESIAN_POINT ( 'NONE',  ( 6.797377311284128254, -286.4689073349238129, -330.6217694938074487 ) ) ;
#756=CARTESIAN_POINT ( 'NONE',  ( -102.5419994578473109, -292.6735454659420270, -230.8212709184644780 ) ) ;
#757=CARTESIAN_POINT ( 'NONE',  ( 23.18044467625053073, -293.0467460412842229, -311.8176801205185598 ) ) ;
#758=CARTESIAN_POINT ( 'NONE',  ( -23.51899185931068814, -294.5374246873147968, -342.1136448299192807 ) ) ;
#759=CARTESIAN_POINT ( 'NONE',  ( -88.45374369700220996, -292.4348123581069672, -213.1854980804716035 ) ) ;
#761=CARTESIAN_POINT ( 'NONE',  ( 25.21923189938433651, -281.6825884757689664, -232.4474024143111990 ) ) ;
#762=CARTESIAN_POINT ( 'NONE',  ( -37.59279624607444958, -296.9694114674621801, -193.6706396809427133 ) ) ;
#763=CARTESIAN_POINT ( 'NONE',  ( -31.82579664469638914, -289.6358137486776627, -347.1135885367444303 ) ) ;
#764=CARTESIAN_POINT ( 'NONE',  ( -38.73399144683423145, -281.2090305365150584, -346.1131279147828081 ) ) ;
#765=CARTESIAN_POINT ( 'NONE',  ( 21.47561144938456579, -288.5546550054625072, -320.0226539073504455 ) ) ;
#766=CARTESIAN_POINT ( 'NONE',  ( -69.99569326733218588, -285.9430435095978851, -205.0340450781253878 ) ) ;
#767=CARTESIAN_POINT ( 'NONE',  ( 153.3814170968207407, 207.2574094408751080, -217.2232996818673882 ) ) ;
#768=CARTESIAN_POINT ( 'NONE',  ( -112.6840901989520205, -268.7463710152937892, -295.7251649536935361 ) ) ;
#769=CARTESIAN_POINT ( 'NONE',  ( 192.8699606740408683, 275.8991237878555012, -123.9883993914645401 ) ) ;
#771=CARTESIAN_POINT ( 'NONE',  ( -108.1262211969130362, -277.9935815721493100, -251.8145494874757162 ) ) ;
#772=CARTESIAN_POINT ( 'NONE',  ( -95.02559501780957874, -278.1079005459940845, -225.0994072091617113 ) ) ;
#773=CARTESIAN_POINT ( 'NONE',  ( -36.93558084685878384, -273.7238594976064405, -193.3702845615455601 ) ) ;
#774=CARTESIAN_POINT ( 'NONE',  ( -96.94098799420999057, -247.8563818616659944, -332.2110617558730610 ) ) ;
#775=CARTESIAN_POINT ( 'NONE',  ( -105.6406974281751303, -277.5723512479806914, -235.9817885254865928 ) ) ;
#776=CARTESIAN_POINT ( 'NONE',  ( -85.95157403567156962, -281.7497591143824707, -327.0085094357900743 ) ) ;
#777=CARTESIAN_POINT ( 'NONE',  ( -33.46383412104373889, -296.7641339003956205, -346.2617194651964496 ) ) ;
#779=CARTESIAN_POINT ( 'NONE',  ( -20.06368573482255968, -292.7724513813253111, -199.3196609204650827 ) ) ;
#780=CARTESIAN_POINT ( 'NONE',  ( -39.99255981794238579, -287.7708479432874356, -343.8563621197477573 ) ) ;
#781=CARTESIAN_POINT ( 'NONE',  ( -113.7622917854316569, -273.3107105573316744, -261.8050699941366020 ) ) ;
#782=CARTESIAN_POINT ( 'NONE',  ( -86.10186548931618233, -297.5199146281921685, -216.0339030858638694 ) ) ;
#785=CARTESIAN_POINT ( 'NONE',  ( -99.08665254665626776, -281.0595455446512005, -226.8079889331963841 ) ) ;
#787=CARTESIAN_POINT ( 'NONE',  ( -37.02071557574380023, -281.1359384565927826, -197.0527075262578762 ) ) ;
#788=CARTESIAN_POINT ( 'NONE',  ( -110.4592604946704597, -280.0496039754244180, -291.0443571144713246 ) ) ;
#789=CARTESIAN_POINT ( 'NONE',  ( -37.55320148959520310, -282.1136453882205615, -343.6085773246091435 ) ) ;
#790=CARTESIAN_POINT ( 'NONE',  ( 15.96154643515947136, -273.3042590122290108, -219.4003769238387349 ) ) ;
#795=CARTESIAN_POINT ( 'NONE',  ( 29.80144657926215146, -275.8684020394861705, -232.8892292355113227 ) ) ;
#797=CARTESIAN_POINT ( 'NONE',  ( -4.837950822480131308, -278.6242992889652328, -337.9659741168057963 ) ) ;
#798=CARTESIAN_POINT ( 'NONE',  ( -70.06527597014458308, -276.0494973529995946, -339.4245148474988696 ) ) ;
#801=CARTESIAN_POINT ( 'NONE',  ( 36.81162679258469694, -283.7042654170799665, -283.8378040925136929 ) ) ;
#802=CARTESIAN_POINT ( 'NONE',  ( -95.23591547362887866, -290.3777209622477926, -225.6301269694029656 ) ) ;
#803=CARTESIAN_POINT ( 'NONE',  ( 12.01850982276712010, -286.0659370170184843, -211.3265329020892409 ) ) ;
#804=CARTESIAN_POINT ( 'NONE',  ( -26.61780063314323641, -281.1538624164415978, -343.6454429888399318 ) ) ;
#805=CARTESIAN_POINT ( 'NONE',  ( -61.74712069394157510, -281.9502078603786686, -339.8392114669903208 ) ) ;
#806=CARTESIAN_POINT ( 'NONE',  ( 35.40842217358378718, -285.4279737154595864, -254.5898178880433704 ) ) ;
#807=CARTESIAN_POINT ( 'NONE',  ( 32.61443292740886335, -283.0520645491343998, -292.7364386427111071 ) ) ;
#808=CARTESIAN_POINT ( 'NONE',  ( -72.97167380842988393, -271.5802567225570670, -204.3071389892957086 ) ) ;
#809=CARTESIAN_POINT ( 'NONE',  ( -80.46847368171820847, -283.8785524581387563, -207.4760904748688120 ) ) ;
#810=CARTESIAN_POINT ( 'NONE',  ( -78.36125111334239079, -297.6042968928582013, -333.1496287471148321 ) ) ;
#811=CARTESIAN_POINT ( 'NONE',  ( -110.4021442392933778, -279.4178257768415961, -276.1092480629901047 ) ) ;
#812=CARTESIAN_POINT ( 'NONE',  ( -15.95994241996441154, -288.3280766862233122, -198.2456266740734065 ) ) ;
#815=CARTESIAN_POINT ( 'NONE',  ( 21.08002887603609921, -294.8165126384732275, -222.4422721897455801 ) ) ;
#816=CARTESIAN_POINT ( 'NONE',  ( -111.0125257249000441, -276.3706251386071244, -284.4864801008928339 ) ) ;
#817=CARTESIAN_POINT ( 'NONE',  ( 14.48723273717265236, -287.5424470332873739, -327.1599286408305147 ) ) ;
#818=CARTESIAN_POINT ( 'NONE',  ( 32.56533995485899169, -291.6392899356585531, -246.5492913139481175 ) ) ;
#819=CARTESIAN_POINT ( 'NONE',  ( -91.34150605533277201, -276.5251455691686715, -320.2875890802395134 ) ) ;
#820=CARTESIAN_POINT ( 'NONE',  ( -83.14016282443174077, -293.8260117241777039, -328.8506944977291369 ) ) ;
#821=CARTESIAN_POINT ( 'NONE',  ( -1.027474884110952891, -293.8600899611792556, -206.4519417833921295 ) ) ;
#824=CARTESIAN_POINT ( 'NONE',  ( -85.96850898010794140, -294.1919638546614806, -329.1670803653922235 ) ) ;
#825=CARTESIAN_POINT ( 'NONE',  ( 35.55258103312795726, -289.3037453561979646, -281.9684635509040049 ) ) ;
#826=CARTESIAN_POINT ( 'NONE',  ( -104.2741155191697828, -288.3207402773603576, -306.3336878296482837 ) ) ;
#827=CARTESIAN_POINT ( 'NONE',  ( 19.98382587014834399, -289.6245471116602062, -316.5039287782337283 ) ) ;
#829=CARTESIAN_POINT ( 'NONE',  ( -94.22339290928100297, -290.7056025044375929, -316.3727986070716724 ) ) ;
#831=CARTESIAN_POINT ( 'NONE',  ( 22.98430296411414275, -289.3917007370027363, -317.5922224971516243 ) ) ;
#832=CARTESIAN_POINT ( 'NONE',  ( -105.9117318151228204, -276.9818752618339204, -238.9856587709358280 ) ) ;
#833=CARTESIAN_POINT ( 'NONE',  ( -33.92045958425376995, -280.4273695767720369, -193.4583260649926331 ) ) ;
#834=CARTESIAN_POINT ( 'NONE',  ( 29.74138991309138191, -281.7101127769357731, -308.2269072033902830 ) ) ;
#835=CARTESIAN_POINT ( 'NONE',  ( 35.96011129240598336, -285.7564829485111773, -286.2908819176259954 ) ) ;
#836=CARTESIAN_POINT ( 'NONE',  ( -111.3408027809598622, -274.2966735324315550, -270.3833299183785357 ) ) ;
#837=CARTESIAN_POINT ( 'NONE',  ( -84.19936477283708598, -277.5398685475452112, -212.7166139035312824 ) ) ;
#838=CARTESIAN_POINT ( 'NONE',  ( -31.80989545341614289, -280.9821973052985413, -345.1697616508848228 ) ) ;
#840=CARTESIAN_POINT ( 'NONE',  ( -86.66195202741687353, -276.2028282026039960, -328.6558689310012937 ) ) ;
#842=CARTESIAN_POINT ( 'NONE',  ( -97.80922045200648540, -282.8396864420637371, -317.5328414729910946 ) ) ;
#843=CARTESIAN_POINT ( 'NONE',  ( -69.57128714561385152, -274.4194747542948676, -204.6811709041430447 ) ) ;
#844=CARTESIAN_POINT ( 'NONE',  ( -100.4056891817341750, -292.6744678486936664, -232.0287074297657739 ) ) ;
#845=CARTESIAN_POINT ( 'NONE',  ( 75.46536863027608888, -300.7518833175248005, -193.8295958960177359 ) ) ;
#846=CARTESIAN_POINT ( 'NONE',  ( 3.142303339223668335, -276.1582845308063270, -331.1322702669907585 ) ) ;
#847=CARTESIAN_POINT ( 'NONE',  ( -38.34415815245513670, -297.0648776346940849, -345.3544225554792888 ) ) ;
#848=CARTESIAN_POINT ( 'NONE',  ( -91.59702342025792632, -289.9655573783689988, -325.0745681992650020 ) ) ;
#849=CARTESIAN_POINT ( 'NONE',  ( 23.44806425252539128, -279.0242799450177813, -225.4844119210102917 ) ) ;
#850=CARTESIAN_POINT ( 'NONE',  ( -50.56426823603852228, -291.7210690224612790, -194.5049139045978563 ) ) ;
#851=CARTESIAN_POINT ( 'NONE',  ( -56.13750644488317931, -288.3588724156700209, -341.1960910039237547 ) ) ;
#852=CARTESIAN_POINT ( 'NONE',  ( -78.40383310051349497, -293.6046204358681848, -333.1217894481948747 ) ) ;
#855=CARTESIAN_POINT ( 'NONE',  ( -103.6095035000222992, -290.4747574026792449, -239.5947942224024985 ) ) ;
#857=CARTESIAN_POINT ( 'NONE',  ( 7.397043513501998291, -287.5866334202389680, -207.9156505405056237 ) ) ;
#858=CARTESIAN_POINT ( 'NONE',  ( -6.941161984400275209, -291.1233781216987495, -333.4151289067050357 ) ) ;
#859=CARTESIAN_POINT ( 'NONE',  ( -74.50299741682368904, -294.5923945951759606, -337.5910194094132066 ) ) ;
#860=CARTESIAN_POINT ( 'NONE',  ( -44.35720491379382224, -284.4541675825812490, -346.5986523463424192 ) ) ;
#861=CARTESIAN_POINT ( 'NONE',  ( -110.2280873567793691, -284.4500841960836510, -265.4630893970663692 ) ) ;
#862=CARTESIAN_POINT ( 'NONE',  ( 27.20785419408808536, -277.3449904248215603, -305.6044022578221302 ) ) ;
#863=CARTESIAN_POINT ( 'NONE',  ( 11.34570631553869369, -292.3934316537889231, -326.9418855063963747 ) ) ;
#866=CARTESIAN_POINT ( 'NONE',  ( 34.51321214708612217, -274.1499004116412834, -255.3330016623347944 ) ) ;
#868=CARTESIAN_POINT ( 'NONE',  ( 138.4517698930976621, 181.0451598467585939, -241.7086681466011271 ) ) ;
#869=CARTESIAN_POINT ( 'NONE',  ( 28.08571317074149576, -293.7505785399827118, -311.0198277226323853 ) ) ;
#870=CARTESIAN_POINT ( 'NONE',  ( -6.440618138260185255, -288.3813296097144416, -202.6238822446383381 ) ) ;
#871=CARTESIAN_POINT ( 'NONE',  ( -113.6343124262126594, -297.5338059234313164, -278.1668734224252262 ) ) ;
#872=CARTESIAN_POINT ( 'NONE',  ( 19.58935568490491264, -287.5559108559137371, -224.4855621633024896 ) ) ;
#873=CARTESIAN_POINT ( 'NONE',  ( -113.0025450158317284, -277.7736261043972377, -257.3897354765216505 ) ) ;
#874=CARTESIAN_POINT ( 'NONE',  ( -30.59162539493526367, -295.6203245123036822, -346.9623534663205646 ) ) ;
#875=CARTESIAN_POINT ( 'NONE',  ( -12.64904773237395652, -286.8742108251241234, -342.0441420440407114 ) ) ;
#876=CARTESIAN_POINT ( 'NONE',  ( 37.76423380660313001, -294.0973076432025550, -287.2979206696631991 ) ) ;
#877=CARTESIAN_POINT ( 'NONE',  ( -67.81388237054360957, -291.9741377566406300, -203.9882533135386211 ) ) ;
#879=CARTESIAN_POINT ( 'NONE',  ( -29.93913374800817451, -125.2961201612322100, -360.6981843053002876 ) ) ;
#880=CARTESIAN_POINT ( 'NONE',  ( 37.60552942728433123, -288.8913044591635639, -256.0216432299667417 ) ) ;
#881=CARTESIAN_POINT ( 'NONE',  ( -2.659677404128736544, -286.1237833571631768, -342.4524372437778652 ) ) ;
#883=CARTESIAN_POINT ( 'NONE',  ( -86.73289319668791109, -278.7350365296442192, -211.3525748638704442 ) ) ;
#884=CARTESIAN_POINT ( 'NONE',  ( 25.68802065633659382, -284.0977715745560204, -310.7960192280100387 ) ) ;
#885=CARTESIAN_POINT ( 'NONE',  ( -113.3199147267640257, -283.0245608065034730, -278.4800587053243817 ) ) ;
#886=CARTESIAN_POINT ( 'NONE',  ( -59.13358558329213821, -287.4160669487540645, -341.5938146063364229 ) ) ;
#887=CARTESIAN_POINT ( 'NONE',  ( 28.85658233711649956, -276.9258151481580512, -233.4009841087603263 ) ) ;
#888=CARTESIAN_POINT ( 'NONE',  ( -94.50338430842838022, -297.6865353482889986, -224.8580378279809793 ) ) ;
#889=CARTESIAN_POINT ( 'NONE',  ( 27.58594934652676045, -292.7041980245496688, -304.9029987285169341 ) ) ;
#890=CARTESIAN_POINT ( 'NONE',  ( -72.46765928994960859, -280.2510218501404324, -201.9397621900457693 ) ) ;
#891=CARTESIAN_POINT ( 'NONE',  ( 35.10608272257667295, -275.6756949264022296, -279.7263342099862484 ) ) ;
#892=CARTESIAN_POINT ( 'NONE',  ( -94.01430263645522700, -278.5534451031831509, -224.1863543828957290 ) ) ;
#893=CARTESIAN_POINT ( 'NONE',  ( 4.682238158189504063, -275.6844985772212908, -206.1461012879581745 ) ) ;
#894=CARTESIAN_POINT ( 'NONE',  ( 3.325883021990954092, -275.4399158623971289, -335.4439294335471686 ) ) ;
#895=CARTESIAN_POINT ( 'NONE',  ( 193.6317248235237400, 279.2590636266914998, -125.8091547554434868 ) ) ;
#896=CARTESIAN_POINT ( 'NONE',  ( -13.32075081187344345, -274.7401622057311670, -341.4644680875760514 ) ) ;
#897=CARTESIAN_POINT ( 'NONE',  ( -113.5348082064481758, -298.0583695818863816, -263.9381939740887901 ) ) ;
#898=CARTESIAN_POINT ( 'NONE',  ( -54.49178911615187815, -276.3376638359844151, -195.3683826091709363 ) ) ;
#901=CARTESIAN_POINT ( 'NONE',  ( -41.35353448545914290, -287.0801646925061732, -197.1493095816360892 ) ) ;
#902=CARTESIAN_POINT ( 'NONE',  ( -73.15549711812488454, -287.3445839549407879, -203.2853287080060909 ) ) ;
#903=CARTESIAN_POINT ( 'NONE',  ( -41.32019378768246298, -285.3493596849029927, -197.3550116065925408 ) ) ;
#904=CARTESIAN_POINT ( 'NONE',  ( -77.23738224982504619, -277.9077660217334369, -208.2133749869777830 ) ) ;
#905=CARTESIAN_POINT ( 'NONE',  ( -111.4630947916657249, -286.4768538268582461, -265.4059684462530981 ) ) ;
#906=CARTESIAN_POINT ( 'NONE',  ( -100.0476087580543521, -277.5619938040289867, -231.5510620201579002 ) ) ;
#908=CARTESIAN_POINT ( 'NONE',  ( -41.86196548030189746, -278.1900880526117703, -343.5433876501726331 ) ) ;
#910=CARTESIAN_POINT ( 'NONE',  ( 5.207498729030233697, -275.1372241978257307, -210.9053760634883474 ) ) ;
#911=CARTESIAN_POINT ( 'NONE',  ( 39.18188151753595605, -286.2904574326822740, -265.8571199716314482 ) ) ;
#912=CARTESIAN_POINT ( 'NONE',  ( 38.09420738556068642, -282.1718228230033105, -255.7466498587353101 ) ) ;
#913=CARTESIAN_POINT ( 'NONE',  ( -21.73234326751586210, -283.3495676913545935, -345.6995204175483991 ) ) ;
#917=CARTESIAN_POINT ( 'NONE',  ( 27.85312228968123804, -289.9236316028311649, -308.9608667980314181 ) ) ;
#918=CARTESIAN_POINT ( 'NONE',  ( -105.5567719990287827, -289.6871790054909184, -235.6033080927602441 ) ) ;
#919=CARTESIAN_POINT ( 'NONE',  ( -60.55747184931169613, -296.9404801215839598, -200.9272070775346606 ) ) ;
#920=CARTESIAN_POINT ( 'NONE',  ( 11.06107270794584707, -292.0504144434183900, -210.5390736144928781 ) ) ;
#921=CARTESIAN_POINT ( 'NONE',  ( 35.44096400160235305, -286.1839987365116826, -281.9909303770633642 ) ) ;
#922=CARTESIAN_POINT ( 'NONE',  ( 32.21200578076647503, -288.4475306472336911, -246.9215680932040584 ) ) ;
#923=CARTESIAN_POINT ( 'NONE',  ( -20.19161114001083490, -297.3376638359846424, -345.3538533559490702 ) ) ;
#924=CARTESIAN_POINT ( 'NONE',  ( -36.09388859611323852, -291.0366967872948294, -345.3635108684193256 ) ) ;
#925=CARTESIAN_POINT ( 'NONE',  ( -56.84047808315676065, -287.3027138232282596, -343.0084844117062062 ) ) ;
#926=CARTESIAN_POINT ( 'NONE',  ( -82.93186140916870386, -284.6345351891668543, -327.7406281803029060 ) ) ;
#927=CARTESIAN_POINT ( 'NONE',  ( -108.1301928377422996, -292.2236681056449470, -295.7940793540527693 ) ) ;
#928=CARTESIAN_POINT ( 'NONE',  ( 82.15603094527575934, -298.9910830478302159, -193.4355229634127795 ) ) ;
#931=CARTESIAN_POINT ( 'NONE',  ( -32.06024178434928729, -300.0379246320565585, -194.7993979984996713 ) ) ;
#932=CARTESIAN_POINT ( 'NONE',  ( 18.61126016977251751, -281.4176509715402403, -317.5172562330616870 ) ) ;
#933=CARTESIAN_POINT ( 'NONE',  ( -79.52190423584431755, -281.6218152193807782, -332.3758825793864276 ) ) ;
#934=CARTESIAN_POINT ( 'NONE',  ( -34.87009877148700809, -294.2190133407408439, -347.1598810435261839 ) ) ;
#935=CARTESIAN_POINT ( 'NONE',  ( -102.9180141350952340, -271.2539721410189486, -235.9322371201628528 ) ) ;
#936=CARTESIAN_POINT ( 'NONE',  ( 33.46041149705509810, -273.9310737872325490, -293.3475310819709989 ) ) ;
#937=CARTESIAN_POINT ( 'NONE',  ( -82.25866614509931196, -298.7400811430143790, -212.1269462908238097 ) ) ;
#939=CARTESIAN_POINT ( 'NONE',  ( -94.82974042097328038, -294.1118501104623419, -320.0511495663456571 ) ) ;
#941=CARTESIAN_POINT ( 'NONE',  ( -26.09963061835976816, -296.3314905084831139, -343.0865659981205908 ) ) ;
#943=CARTESIAN_POINT ( 'NONE',  ( -55.83427369241110938, -296.0991008964558091, -341.1993936045574287 ) ) ;
#945=CARTESIAN_POINT ( 'NONE',  ( -112.5091102700940127, -282.6490287972261513, -264.3537110432848749 ) ) ;
#946=CARTESIAN_POINT ( 'NONE',  ( -110.0992216245961401, -296.4658981593526050, -276.8996432020963425 ) ) ;
#947=CARTESIAN_POINT ( 'NONE',  ( -92.43373764308211094, -283.8142233278933872, -324.1557961807400829 ) ) ;
#948=CARTESIAN_POINT ( 'NONE',  ( 25.53737957532825575, -284.0342829684607864, -312.2602293522240871 ) ) ;
#949=CARTESIAN_POINT ( 'NONE',  ( 12.06725818327686461, -286.3840178553754185, -211.2619120057407827 ) ) ;
#950=CARTESIAN_POINT ( 'NONE',  ( 16.20471157591834910, -290.8135480297377740, -218.0105845512304086 ) ) ;
#951=CARTESIAN_POINT ( 'NONE',  ( -112.2420342695258313, -277.9642507728015630, -253.2118099222299179 ) ) ;
#952=CARTESIAN_POINT ( 'NONE',  ( -95.99890600148557951, -281.4094976428775681, -317.0979686699210447 ) ) ;
#954=CARTESIAN_POINT ( 'NONE',  ( 35.14898454146587881, -286.4989941086593035, -281.9402881070710691 ) ) ;
#955=CARTESIAN_POINT ( 'NONE',  ( -54.44610676298083263, -288.1871189736680208, -345.1747707523663280 ) ) ;
#956=CARTESIAN_POINT ( 'NONE',  ( -100.5928439528197202, -298.6709374801468471, -232.2388944273133973 ) ) ;
#957=CARTESIAN_POINT ( 'NONE',  ( -110.7760353280859675, -280.2442397757020558, -249.2422944540280412 ) ) ;
#958=CARTESIAN_POINT ( 'NONE',  ( -22.44783362419774519, -292.8824680474103275, -344.2297821128346982 ) ) ;
#959=CARTESIAN_POINT ( 'NONE',  ( 35.72392568591476447, -281.2314915197200094, -271.3182695534003983 ) ) ;
#960=CARTESIAN_POINT ( 'NONE',  ( 33.41740802365017515, -294.1071294063391406, -300.8626818259278366 ) ) ;
#961=CARTESIAN_POINT ( 'NONE',  ( -2.857853123212670710, -284.5841079123286477, -203.1143665305021102 ) ) ;
#962=CARTESIAN_POINT ( 'NONE',  ( -94.40124125525481702, -281.2264783105441666, -221.6668586528346907 ) ) ;
#963=CARTESIAN_POINT ( 'NONE',  ( -110.6093951094849928, -295.6325305761101845, -268.7156878205362318 ) ) ;
#966=CARTESIAN_POINT ( 'NONE',  ( 35.35669359156745628, -283.3135614387476267, -253.4262321628382040 ) ) ;
#968=CARTESIAN_POINT ( 'NONE',  ( -54.42813229853333468, -277.3380690714490697, -195.3538533559490702 ) ) ;
#969=CARTESIAN_POINT ( 'NONE',  ( -35.51735102929995946, -273.2716381086009392, -193.5311515974589440 ) ) ;
#970=CARTESIAN_POINT ( 'NONE',  ( -106.0332877464310286, -290.0564094396924588, -295.0687239970229712 ) ) ;
#971=CARTESIAN_POINT ( 'NONE',  ( -11.51815736585606054, -281.9146998990236739, -201.2864930753476642 ) ) ;
#972=CARTESIAN_POINT ( 'NONE',  ( -4.975394387236288907, -276.0856964431934557, -204.0232223557427460 ) ) ;
#973=CARTESIAN_POINT ( 'NONE',  ( 36.42256047748497139, -283.3939899960176376, -289.4732679058714666 ) ) ;
#974=CARTESIAN_POINT ( 'NONE',  ( 5.813239184487858147, -281.2472027869869748, -329.7309901121471398 ) ) ;
#975=CARTESIAN_POINT ( 'NONE',  ( -37.79701941603578064, -279.0579763704753304, -345.3725346836218932 ) ) ;
#977=CARTESIAN_POINT ( 'NONE',  ( 4.864935244613048049, -274.4383479087302931, -205.8959925199068550 ) ) ;
#978=CARTESIAN_POINT ( 'NONE',  ( 24.52468685203869114, -294.9084711916231072, -228.9622730710885037 ) ) ;
#981=CARTESIAN_POINT ( 'NONE',  ( 22.18623702242076945, -292.3289950001711759, -317.2512136965749505 ) ) ;
#982=CARTESIAN_POINT ( 'NONE',  ( -0.5098349863465404530, -274.0635525867834872, -207.2481611531588044 ) ) ;
#984=CARTESIAN_POINT ( 'NONE',  ( 8.419526694714949855, -294.1856584809298738, -209.2327734719434886 ) ) ;
#985=CARTESIAN_POINT ( 'NONE',  ( -37.37352853689063892, -282.5519495502701943, -195.3611179825600175 ) ) ;
#986=CARTESIAN_POINT ( 'NONE',  ( -16.74818689177746478, -293.5175093448845587, -196.5782207085586606 ) ) ;
#987=CARTESIAN_POINT ( 'NONE',  ( -2.490413321436029559, -290.5905754256617115, -336.6409961592946729 ) ) ;
#988=CARTESIAN_POINT ( 'NONE',  ( 35.95524251878263300, -273.7461268672862502, -285.4470925500735348 ) ) ;
#989=CARTESIAN_POINT ( 'NONE',  ( -32.29905878450974654, -278.9083651082324877, -344.6810802384226236 ) ) ;
#990=CARTESIAN_POINT ( 'NONE',  ( 34.12595542525693304, -291.9026829951419018, -291.2320673009564871 ) ) ;
#991=CARTESIAN_POINT ( 'NONE',  ( -4.219348060625711661, -282.3445218360288322, -202.2056929960885157 ) ) ;
#994=CARTESIAN_POINT ( 'NONE',  ( -24.06581367699070739, -282.5446068761607421, -342.1652844746584492 ) ) ;
#995=CARTESIAN_POINT ( 'NONE',  ( -74.86872700455558061, -280.6441707290950376, -203.4790219939885105 ) ) ;
#997=CARTESIAN_POINT ( 'NONE',  ( 0.6579846690457067382, -281.3521927483833451, -336.8896722809365656 ) ) ;
#998=CARTESIAN_POINT ( 'NONE',  ( -14.64778039991939096, -277.7064287355931356, -343.7503030558007140 ) ) ;
#1001=CARTESIAN_POINT ( 'NONE',  ( 27.89961750840676302, -276.5497980251693093, -230.6839122871389236 ) ) ;
#1002=CARTESIAN_POINT ( 'NONE',  ( -105.5795714935544112, -286.8376638359844719, -285.9686137636504668 ) ) ;
#1004=CARTESIAN_POINT ( 'NONE',  ( -67.65030268694809479, -299.6546725967230032, -201.7439321594510773 ) ) ;
#1005=CARTESIAN_POINT ( 'NONE',  ( -79.58310737088281428, -275.6456418185090342, -331.9668237205792138 ) ) ;
#1006=CARTESIAN_POINT ( 'NONE',  ( -111.5705844000524536, -292.1063541941880430, -286.6106335787735588 ) ) ;
#1007=CARTESIAN_POINT ( 'NONE',  ( -17.39682783762583185, -291.6648620706661745, -199.9799727888749601 ) ) ;
#1008=CARTESIAN_POINT ( 'NONE',  ( -3.093761974300191397, -288.1195746266095057, -339.2713484225133129 ) ) ;
#1010=CARTESIAN_POINT ( 'NONE',  ( 33.91993294284144156, -291.7732104812580474, -242.6397112975752464 ) ) ;
#1011=CARTESIAN_POINT ( 'NONE',  ( -110.8947407714575348, -282.8733013534049974, -276.3935823160416589 ) ) ;
#1012=CARTESIAN_POINT ( 'NONE',  ( -110.1455382575282300, -292.2235340083572623, -284.9335032823274219 ) ) ;
#1013=CARTESIAN_POINT ( 'NONE',  ( -100.1906034999029202, -283.5584432064873113, -231.7837677653867274 ) ) ;
#1015=CARTESIAN_POINT ( 'NONE',  ( -71.62417836667094662, -284.8303029174610401, -335.3684649896103451 ) ) ;
#1016=CARTESIAN_POINT ( 'NONE',  ( -62.67465757400178461, -290.3150765332896412, -342.8815348908123042 ) ) ;
#1018=CARTESIAN_POINT ( 'NONE',  ( 35.49091247449603514, -282.1287150791714566, -276.7502876014257254 ) ) ;
#1019=CARTESIAN_POINT ( 'NONE',  ( 26.17232062719289232, -291.7788378357195143, -227.4428137465853865 ) ) ;
#1020=CARTESIAN_POINT ( 'NONE',  ( 2.648228718991627595, -287.3769849079112078, -204.7488903786906462 ) ) ;
#1021=CARTESIAN_POINT ( 'NONE',  ( 14.56681859312259952, -288.8374182808695423, -327.2226890994894575 ) ) ;
#1022=CARTESIAN_POINT ( 'NONE',  ( -30.53339763175301869, -286.3071789976789319, -197.6284991167072178 ) ) ;
#1025=CARTESIAN_POINT ( 'NONE',  ( -50.23365427689127216, -297.0752956370846505, -345.0741110681527175 ) ) ;
#1026=CARTESIAN_POINT ( 'NONE',  ( -68.04375013930707894, -294.1317519961890525, -340.4373792911929399 ) ) ;
#1027=CARTESIAN_POINT ( 'NONE',  ( -87.68369393546051072, -278.3871389489561352, -217.1018354939701567 ) ) ;
#1028=CARTESIAN_POINT ( 'NONE',  ( -68.12901672938096453, -297.0070944078794923, -199.8384217942894736 ) ) ;
#1029=CARTESIAN_POINT ( 'NONE',  ( 20.74120918621679621, -291.3985485119546865, -224.9856012037972164 ) ) ;
#1030=CARTESIAN_POINT ( 'NONE',  ( -2.455553030725395214, -276.2804968083602262, -205.0853126957729557 ) ) ;
#1031=CARTESIAN_POINT ( 'NONE',  ( -111.3983774615681170, -294.7777569590534767, -271.4560451633701064 ) ) ;
#1032=CARTESIAN_POINT ( 'NONE',  ( 19.64442711626699989, -294.1060809516100107, -224.0842267476853635 ) ) ;
#1033=CARTESIAN_POINT ( 'NONE',  ( 32.64598668094742351, -294.9197028558654665, -292.1773910120720075 ) ) ;
#1035=CARTESIAN_POINT ( 'NONE',  ( -34.93937233869628045, -293.0218790329423086, -345.4893899621767446 ) ) ;
#1036=CARTESIAN_POINT ( 'NONE',  ( -77.72765701591760035, -299.5104587434639143, -207.1024028966750450 ) ) ;
#1037=CARTESIAN_POINT ( 'NONE',  ( -31.84175907741981248, -289.9224447074661839, -343.4403859512186727 ) ) ;
#1038=CARTESIAN_POINT ( 'NONE',  ( -77.95797922591019358, -295.9476078057366522, -331.1050152731499452 ) ) ;
#1039=CARTESIAN_POINT ( 'NONE',  ( -93.74771131835602489, -281.2237479961370923, -220.3934413704049859 ) ) ;
#1040=CARTESIAN_POINT ( 'NONE',  ( -102.9798362976808761, -277.7539956174660460, -230.9525056298894583 ) ) ;
#1041=CARTESIAN_POINT ( 'NONE',  ( 4.814224570445547968, -273.9536928217604554, -205.9847119525065864 ) ) ;
#1042=CARTESIAN_POINT ( 'NONE',  ( 26.38138932523645863, -279.1114354533789310, -231.7815413472453656 ) ) ;
#1043=CARTESIAN_POINT ( 'NONE',  ( -40.94991361842823352, -278.4073685721277798, -194.2335325142391582 ) ) ;
#1044=CARTESIAN_POINT ( 'NONE',  ( -78.87602176098383211, -277.4940363661532388, -207.6494441230378243 ) ) ;
#1045=CARTESIAN_POINT ( 'NONE',  ( -96.74636351259668743, -271.7312411991802037, -226.8430752619213422 ) ) ;
#1046=CARTESIAN_POINT ( 'NONE',  ( 36.52757507304578155, -277.3847850654564695, -257.3137226342531108 ) ) ;
#1048=CARTESIAN_POINT ( 'NONE',  ( -80.95740930335308860, -289.4832423238537444, -208.9113278011794819 ) ) ;
#1049=CARTESIAN_POINT ( 'NONE',  ( -102.3012601845920813, -290.0091174574806132, -311.8023811898784174 ) ) ;
#1050=CARTESIAN_POINT ( 'NONE',  ( -73.09581931445028147, -275.5799314238806232, -204.1846322639948710 ) ) ;
#1051=CARTESIAN_POINT ( 'NONE',  ( -111.0917832501413613, -270.7306310493452770, -256.4483517006355555 ) ) ;
#1052=CARTESIAN_POINT ( 'NONE',  ( -63.13758041765268558, -284.9216999928629548, -197.9820368860418398 ) ) ;
#1054=CARTESIAN_POINT ( 'NONE',  ( 7.283460102669957692, -280.4442333741813513, -330.7041645467697322 ) ) ;
#1056=CARTESIAN_POINT ( 'NONE',  ( 30.22726478279970408, -291.9627847652411106, -241.5680615429741920 ) ) ;
#1057=CARTESIAN_POINT ( 'NONE',  ( -19.49636631882197335, -284.4237012843408934, -198.3027420730902861 ) ) ;
#1060=CARTESIAN_POINT ( 'NONE',  ( -5.160997246936801730, -290.4755195668607257, -202.6018229802685084 ) ) ;
#1061=CARTESIAN_POINT ( 'NONE',  ( -56.79160173907078502, -278.9071419925335817, -341.6050690812330686 ) ) ;
#1062=CARTESIAN_POINT ( 'NONE',  ( -95.95652540879055437, -285.0894613208590158, -319.6998732974388417 ) ) ;
#1063=CARTESIAN_POINT ( 'NONE',  ( 23.33833486314566485, -273.0219709064349445, -225.3361520858668996 ) ) ;
#1064=CARTESIAN_POINT ( 'NONE',  ( -89.66285601298389452, -285.2889704125552157, -219.3818339802222681 ) ) ;
#1065=CARTESIAN_POINT ( 'NONE',  ( 34.40420059604100800, -276.7625747367278564, -253.9371706092239265 ) ) ;
#1066=CARTESIAN_POINT ( 'NONE',  ( -32.39946055657536306, -277.7912239715001306, -343.4055505056790594 ) ) ;
#1067=CARTESIAN_POINT ( 'NONE',  ( -111.8361580510258761, -286.6639379119470732, -261.6676499405724599 ) ) ;
#1070=CARTESIAN_POINT ( 'NONE',  ( -105.9586663602423329, -295.9342305605439378, -305.4172663811372672 ) ) ;
#1071=CARTESIAN_POINT ( 'NONE',  ( -28.96403834222452645, -290.9253240127049480, -344.5343044090064382 ) ) ;
#1073=CARTESIAN_POINT ( 'NONE',  ( -99.86837403722181250, -280.4090924074130839, -320.2651865833026363 ) ) ;
#1074=CARTESIAN_POINT ( 'NONE',  ( -74.84472348819954846, -278.4851765789962883, -203.4655594688400697 ) ) ;
#1075=CARTESIAN_POINT ( 'NONE',  ( 16.97682621455858509, -292.6941502471668173, -323.8771238473130438 ) ) ;
#1076=CARTESIAN_POINT ( 'NONE',  ( 15.51342248968685134, -288.3367469005635257, -219.0089635461066848 ) ) ;
#1077=CARTESIAN_POINT ( 'NONE',  ( -109.7515702377337732, -280.1129305147493938, -285.6838046556247832 ) ) ;
#1078=CARTESIAN_POINT ( 'NONE',  ( 33.50290191486368485, -289.3452869432337025, -299.1316415469081562 ) ) ;
#1079=CARTESIAN_POINT ( 'NONE',  ( -51.36761110440766487, -285.2315219378303368, -344.0909291930940412 ) ) ;
#1080=CARTESIAN_POINT ( 'NONE',  ( -98.80214108853407140, -278.1008545729783350, -316.7682528913188094 ) ) ;
#1081=CARTESIAN_POINT ( 'NONE',  ( -63.63577030268957913, -295.7279645418488485, -200.4460907883798768 ) ) ;
#1082=CARTESIAN_POINT ( 'NONE',  ( -88.92987249621317858, -279.1839301068368400, -213.1976639563723666 ) ) ;
#1083=CARTESIAN_POINT ( 'NONE',  ( -108.3854495593476059, -274.6950023225707014, -248.6522826635056731 ) ) ;
#1085=CARTESIAN_POINT ( 'NONE',  ( -85.28047601435908120, -286.1948066931273615, -330.5268031993605859 ) ) ;
#1086=CARTESIAN_POINT ( 'NONE',  ( -10.68186013637759224, -272.6348704612724987, -199.1487784743132465 ) ) ;
#1088=CARTESIAN_POINT ( 'NONE',  ( -92.25054720890470605, -278.7473530858525805, -222.1445057983821698 ) ) ;
#1089=CARTESIAN_POINT ( 'NONE',  ( 8.018354576881192131, -277.6528932049073433, -332.1558390401979182 ) ) ;
#1090=CARTESIAN_POINT ( 'NONE',  ( -95.76787336223216585, -298.6020088580048082, -225.5995783673533026 ) ) ;
#1091=CARTESIAN_POINT ( 'NONE',  ( -108.0152221341671321, -283.2267562136801757, -300.4650276262655666 ) ) ;
#1092=CARTESIAN_POINT ( 'NONE',  ( 35.52319090334380292, -289.4812808199564529, -283.3488687464272289 ) ) ;
#1093=CARTESIAN_POINT ( 'NONE',  ( -51.68940292160099403, -299.3920739648045810, -195.3616105337451643 ) ) ;
#1094=CARTESIAN_POINT ( 'NONE',  ( -111.8914892694033369, -297.9786938558639804, -252.7447148475994254 ) ) ;
#1095=CARTESIAN_POINT ( 'NONE',  ( -4.719850195966968975, -296.6216490810683695, -337.7239481761257593 ) ) ;
#1096=CARTESIAN_POINT ( 'NONE',  ( 26.71855632994155982, -279.0314419247802107, -231.5784512824415913 ) ) ;
#1097=CARTESIAN_POINT ( 'NONE',  ( -0.8980460531410958680, -272.5585906576740172, -205.2027395754095949 ) ) ;
#1098=CARTESIAN_POINT ( 'NONE',  ( 28.00192510623821462, -288.6345080858802703, -231.0592566860217119 ) ) ;
#1099=CARTESIAN_POINT ( 'NONE',  ( -100.5775226989478881, -288.9642007296278621, -307.5482832304992371 ) ) ;
#1100=CARTESIAN_POINT ( 'NONE',  ( 198.9745609140036606, 284.0578480540463602, -111.6648769956217535 ) ) ;
#1102=CARTESIAN_POINT ( 'NONE',  ( 23.66076176483710825, -286.7443653981940770, -316.3753107662619186 ) ) ;
#1103=CARTESIAN_POINT ( 'NONE',  ( -74.73037293595314168, -289.2313689901456542, -333.0988087027815823 ) ) ;
#1105=CARTESIAN_POINT ( 'NONE',  ( -83.10249885895767363, -286.5220519591247808, -208.7526911711092907 ) ) ;
#1106=CARTESIAN_POINT ( 'NONE',  ( -56.60166329816466657, -277.6404986654090976, -340.8489998805523555 ) ) ;
#1107=CARTESIAN_POINT ( 'NONE',  ( -0.9384164133903355465, -291.4442618767709519, -202.8607961676685534 ) ) ;
#1108=CARTESIAN_POINT ( 'NONE',  ( 36.07591863791223119, -281.9158374490495476, -247.4882947784958276 ) ) ;
#1110=CARTESIAN_POINT ( 'NONE',  ( 34.95844376996689107, -283.3842659259722723, -294.9262075890190999 ) ) ;
#1111=CARTESIAN_POINT ( 'NONE',  ( 4.537755288195992165, -282.8372464690514221, -335.0140232264483870 ) ) ;
#1112=CARTESIAN_POINT ( 'NONE',  ( -1.959548566176730233, -280.8678831060333891, -206.4847464695805570 ) ) ;
#1113=CARTESIAN_POINT ( 'NONE',  ( 174.3702828278471202, 243.3002394640316766, -179.7950274582404120 ) ) ;
#1114=CARTESIAN_POINT ( 'NONE',  ( -100.7144291363231048, -280.0150311131046692, -310.2564250008069280 ) ) ;
#1115=CARTESIAN_POINT ( 'NONE',  ( 4.499940650622777483, -57.89452529514181833, -353.9072000911820055 ) ) ;
#1116=CARTESIAN_POINT ( 'NONE',  ( 191.9139817438699822, 276.9408567967533372, -124.2323592714584777 ) ) ;
#1117=CARTESIAN_POINT ( 'NONE',  ( -108.6901069843859489, -271.9623749435439208, -254.1745010833050742 ) ) ;
#1118=CARTESIAN_POINT ( 'NONE',  ( 38.79193668294810493, -292.9164059715525354, -258.9040720017960098 ) ) ;
#1119=CARTESIAN_POINT ( 'NONE',  ( -107.0837456695891348, -264.9657348211522958, -305.5179930709127802 ) ) ;
#1120=CARTESIAN_POINT ( 'NONE',  ( -91.80616674160452817, -271.9798102298358344, -216.6310505271245859 ) ) ;
#1121=CARTESIAN_POINT ( 'NONE',  ( -10.45139258062658172, -287.0953617368729738, -339.1425665127841285 ) ) ;
#1122=CARTESIAN_POINT ( 'NONE',  ( -8.733334960409219860, -296.5342515798746490, -338.8762476456487889 ) ) ;
#1123=CARTESIAN_POINT ( 'NONE',  ( 33.50019461619996264, -288.6105727994026324, -250.7991797362542172 ) ) ;
#1125=CARTESIAN_POINT ( 'NONE',  ( 4.110360476094063742, -295.4498316236593496, -335.0344413311789822 ) ) ;
#1126=CARTESIAN_POINT ( 'NONE',  ( -46.73899239170622621, -286.4221153722847930, -197.8556285555808643 ) ) ;
#1127=CARTESIAN_POINT ( 'NONE',  ( -52.47113154244657807, -272.7832085550333545, -195.1231704729238743 ) ) ;
#1128=CARTESIAN_POINT ( 'NONE',  ( -69.56478962876855121, -292.4415673326432170, -200.5912948374864584 ) ) ;
#1129=CARTESIAN_POINT ( 'NONE',  ( 25.66786172475784866, -294.6290315133653053, -314.5352401015075543 ) ) ;
#1130=CARTESIAN_POINT ( 'NONE',  ( -108.1089997933592315, -290.9559001142337138, -252.3940989468879650 ) ) ;
#1132=CARTESIAN_POINT ( 'NONE',  ( -80.44930343749901169, -275.3935366908764877, -208.2408831466813979 ) ) ;
#1133=CARTESIAN_POINT ( 'NONE',  ( -1.473759650709204561, -273.3119385549804292, -202.6743425727264594 ) ) ;
#1136=CARTESIAN_POINT ( 'NONE',  ( -25.78540478833620497, -276.4163586253898757, -346.4267405798486266 ) ) ;
#1137=CARTESIAN_POINT ( 'NONE',  ( -66.10637053541185537, -272.0691433264092325, -202.3976413741297904 ) ) ;
#1138=CARTESIAN_POINT ( 'NONE',  ( -32.36095606487933196, -275.1284053316981613, -344.4798563065289727 ) ) ;
#1139=CARTESIAN_POINT ( 'NONE',  ( -93.15803736730549645, -274.3051355363830908, -222.8152951516119629 ) ) ;
#1140=CARTESIAN_POINT ( 'NONE',  ( -105.6400026229400311, -273.8471441581478985, -243.7872833854606824 ) ) ;
#1141=CARTESIAN_POINT ( 'NONE',  ( -87.38607253133439201, -275.1259472180560124, -213.1112975050200475 ) ) ;
#1143=CARTESIAN_POINT ( 'NONE',  ( 31.07062864848332850, -273.1578201555006444, -238.6430976653437597 ) ) ;
#1144=CARTESIAN_POINT ( 'NONE',  ( -108.3961317111346858, -296.9765516566779411, -287.5941142982170504 ) ) ;
#1145=CARTESIAN_POINT ( 'NONE',  ( -6.534635463886656837, -293.2141614698999206, -337.1914979426683772 ) ) ;
#1147=CARTESIAN_POINT ( 'NONE',  ( 16.91627887158795929, -276.7969609196704823, -324.9845656149531692 ) ) ;
#1148=CARTESIAN_POINT ( 'NONE',  ( -4.106581969183493719, -274.6697700212742461, -205.3514937019019158 ) ) ;
#1149=CARTESIAN_POINT ( 'NONE',  ( -112.0472043524662951, -283.0292472786928215, -286.8652360616684405 ) ) ;
#1150=CARTESIAN_POINT ( 'NONE',  ( -98.44641521233309334, -299.1465021712577936, -226.5862139532879382 ) ) ;
#1152=CARTESIAN_POINT ( 'NONE',  ( 15.15246052924810805, -286.0141669556790589, -219.4006938889544358 ) ) ;
#1153=CARTESIAN_POINT ( 'NONE',  ( -110.1245732095633940, -276.9668736212078670, -256.9213485965001382 ) ) ;
#1154=CARTESIAN_POINT ( 'NONE',  ( -98.14583666262868178, -276.5548198592151721, -311.8126788427324527 ) ) ;
#1155=CARTESIAN_POINT ( 'NONE',  ( -61.03100585867067451, -285.3596730798511771, -341.5756631663874714 ) ) ;
#1156=CARTESIAN_POINT ( 'NONE',  ( -0.3593866511650910534, -275.7607016248830973, -206.9474036374556078 ) ) ;
#1158=CARTESIAN_POINT ( 'NONE',  ( 21.24893732608056851, -273.2899112099784134, -221.6417417495325424 ) ) ;
#1159=CARTESIAN_POINT ( 'NONE',  ( -8.270145936652498975, -282.4320570641137920, -201.0299653366178916 ) ) ;
#1161=CARTESIAN_POINT ( 'NONE',  ( -75.40291243911637764, -287.4693545276017517, -205.0271372972180757 ) ) ;
#1163=CARTESIAN_POINT ( 'NONE',  ( 33.09993806713283249, -291.2162720582772977, -244.4648538759696521 ) ) ;
#1164=CARTESIAN_POINT ( 'NONE',  ( 82.17077897911026696, -297.8327751790970979, -196.3995604311907641 ) ) ;
#1165=CARTESIAN_POINT ( 'NONE',  ( -69.41728368265411575, -296.4152365729725602, -204.3437911216519467 ) ) ;
#1166=CARTESIAN_POINT ( 'NONE',  ( -49.87432899933946828, -290.0303049508679010, -197.1392690500716185 ) ) ;
#1167=CARTESIAN_POINT ( 'NONE',  ( 193.8665746513534316, 275.1768195097669150, -123.9090917457166938 ) ) ;
#1169=CARTESIAN_POINT ( 'NONE',  ( 37.87673106522297672, -285.8690075228681735, -257.4429778579698791 ) ) ;
#1170=CARTESIAN_POINT ( 'NONE',  ( -29.33785757386130300, -284.5493500736085366, -343.7768735603187906 ) ) ;
#1171=CARTESIAN_POINT ( 'NONE',  ( -110.5216977149730013, -282.5322082173488525, -290.8223488412324969 ) ) ;
#1172=CARTESIAN_POINT ( 'NONE',  ( -10.74601416509237595, -284.1237968329435830, -339.0303281633322285 ) ) ;
#1173=CARTESIAN_POINT ( 'NONE',  ( -93.53955684783119295, -284.6917313239906662, -317.2055693889384997 ) ) ;
#1174=CARTESIAN_POINT ( 'NONE',  ( -103.6954691459158511, -292.0601716343610406, -306.0764387449386845 ) ) ;
#1175=CARTESIAN_POINT ( 'NONE',  ( -52.54560006425432306, -274.1959337515751827, -194.8442124253568863 ) ) ;
#1177=CARTESIAN_POINT ( 'NONE',  ( 21.27231673997742334, -286.2841671170784821, -318.0649201518546647 ) ) ;
#1178=CARTESIAN_POINT ( 'NONE',  ( 38.18236941731774436, -275.7397957691224519, -285.3649481369480441 ) ) ;
#1179=CARTESIAN_POINT ( 'NONE',  ( 36.92927584952963116, -295.4293685446331779, -262.4020301294230535 ) ) ;
#1181=CARTESIAN_POINT ( 'NONE',  ( 21.31550574532285580, -290.6948066931273615, -317.0979686699210447 ) ) ;
#1182=CARTESIAN_POINT ( 'NONE',  ( -53.81639815550146722, -281.9527292216469618, -342.0363733493801988 ) ) ;
#1183=CARTESIAN_POINT ( 'NONE',  ( -59.15783564601671429, -275.3337007900643130, -342.2922284652613030 ) ) ;
#1184=CARTESIAN_POINT ( 'NONE',  ( -60.64083731168902602, -272.2352900528970281, -197.6433630077483201 ) ) ;
#1185=CARTESIAN_POINT ( 'NONE',  ( 13.79671641445455244, -275.6608157164388899, -322.6690945520528544 ) ) ;
#1186=CARTESIAN_POINT ( 'NONE',  ( -9.483153472013412966, -293.9429381436158906, -202.0821335701165538 ) ) ;
#1187=CARTESIAN_POINT ( 'NONE',  ( 20.36089909560774558, -293.8595240299239322, -225.2429429730586889 ) ) ;
#1188=CARTESIAN_POINT ( 'NONE',  ( -98.20179095344455789, -286.8913032155658129, -228.2195495346648499 ) ) ;
#1189=CARTESIAN_POINT ( 'NONE',  ( 38.23643522871735456, -295.1191964814565267, -281.6106401458225719 ) ) ;
#1190=CARTESIAN_POINT ( 'NONE',  ( 37.30647844064418450, -295.0790415012825179, -287.1818011770321846 ) ) ;
#1191=CARTESIAN_POINT ( 'NONE',  ( -108.2995173750590823, -296.1585910187631612, -287.5599210686464744 ) ) ;
#1192=CARTESIAN_POINT ( 'NONE',  ( -99.76145633253106837, -291.9902192124415592, -311.9630231620489553 ) ) ;
#1193=CARTESIAN_POINT ( 'NONE',  ( -33.05662495295239012, -283.1662888241863811, -347.2549276083731797 ) ) ;
#1194=CARTESIAN_POINT ( 'NONE',  ( -36.53468314664176830, -296.1420315690264715, -194.8013716169795941 ) ) ;
#1195=CARTESIAN_POINT ( 'NONE',  ( -87.74833893996564882, -285.2041782759736748, -212.0825361959433906 ) ) ;
#1196=CARTESIAN_POINT ( 'NONE',  ( -41.93312153859111646, -279.0901634900727117, -344.8774589337492671 ) ) ;
#1198=CARTESIAN_POINT ( 'NONE',  ( -101.3300127581286461, -283.8376077873674603, -234.3038855303090315 ) ) ;
#1199=CARTESIAN_POINT ( 'NONE',  ( 35.55434084484616619, -285.7791524868341071, -288.0552444707524273 ) ) ;
#1200=CARTESIAN_POINT ( 'NONE',  ( -95.84822795775885140, -277.3491536565922502, -222.2026946770242262 ) ) ;
#1201=CARTESIAN_POINT ( 'NONE',  ( -90.99921415893403775, -226.8295888252787904, -341.9546587472784154 ) ) ;
#1202=CARTESIAN_POINT ( 'NONE',  ( -97.40295851047305575, -284.6391784208976219, -228.7381206260400290 ) ) ;
#1203=CARTESIAN_POINT ( 'NONE',  ( 32.80316486822700739, -282.3625786447462929, -239.5762737867115959 ) ) ;
#1204=CARTESIAN_POINT ( 'NONE',  ( -71.81158898197851670, -288.5553575073413413, -338.9515471713892794 ) ) ;
#1205=CARTESIAN_POINT ( 'NONE',  ( 16.40555481139226046, -277.9045635920165864, -324.4503068328998552 ) ) ;
#1206=CARTESIAN_POINT ( 'NONE',  ( -37.11152475351090629, -278.3644594539755417, -346.8805982259588632 ) ) ;
#1207=CARTESIAN_POINT ( 'NONE',  ( -46.45435341712889254, -279.7667479160460857, -197.8810193087713856 ) ) ;
#1208=CARTESIAN_POINT ( 'NONE',  ( -10.93134026860996499, -276.3779266610945342, -200.4893906446764618 ) ) ;
#1209=CARTESIAN_POINT ( 'NONE',  ( 6.496230378298051278, -292.6300419999305973, -207.0583862175101615 ) ) ;
#1210=CARTESIAN_POINT ( 'NONE',  ( 13.25253470048357052, -286.3611021679851660, -325.3136617449595747 ) ) ;
#1211=CARTESIAN_POINT ( 'NONE',  ( 12.73723067749040716, -294.3374027913102964, -212.9281909900552705 ) ) ;
#1212=CARTESIAN_POINT ( 'NONE',  ( -6.647956837599817703, -293.5597064423145639, -336.9352886300005707 ) ) ;
#1213=CARTESIAN_POINT ( 'NONE',  ( -41.04453566529495845, -294.7667164892986307, -343.3008888633975744 ) ) ;
#1214=CARTESIAN_POINT ( 'NONE',  ( -111.9587277084514909, -291.4086792588819321, -288.1314329022340530 ) ) ;
#1215=CARTESIAN_POINT ( 'NONE',  ( 0.4455469819851471946, -281.2211471695746923, -207.7244407954254370 ) ) ;
#1216=CARTESIAN_POINT ( 'NONE',  ( -71.28793332262237925, -272.6736272856959999, -201.5100216516559613 ) ) ;
#1217=CARTESIAN_POINT ( 'NONE',  ( 28.82027028128720403, -288.7148236305812361, -309.5517604615333767 ) ) ;
#1218=CARTESIAN_POINT ( 'NONE',  ( 8.443234154030673011, -280.5722833566217105, -330.7270460431906827 ) ) ;
#1220=CARTESIAN_POINT ( 'NONE',  ( -80.52524142950187525, -289.9531053261362104, -334.1509059850862400 ) ) ;
#1222=CARTESIAN_POINT ( 'NONE',  ( -27.83800129034970894, -286.5094488523340601, -197.9610682924675871 ) ) ;
#1224=CARTESIAN_POINT ( 'NONE',  ( 137.1683788224899274, 180.3412242032398467, -239.8556167576348912 ) ) ;
#1225=CARTESIAN_POINT ( 'NONE',  ( 102.7605738203126577, 114.6418858672116414, -279.4648970305247531 ) ) ;
#1226=CARTESIAN_POINT ( 'NONE',  ( -109.2038207892207282, -277.5677594924471805, -284.1546075097517132 ) ) ;
#1227=CARTESIAN_POINT ( 'NONE',  ( -85.31787691779859983, -276.6535200397928520, -325.8586223164987814 ) ) ;
#1228=CARTESIAN_POINT ( 'NONE',  ( -66.21535069744108171, -273.3511189256474836, -198.9883044232203702 ) ) ;
#1229=CARTESIAN_POINT ( 'NONE',  ( -92.67010577559203455, -240.0894200528963154, -339.5335687754159153 ) ) ;
#1230=CARTESIAN_POINT ( 'NONE',  ( -77.16977791118213759, -278.1044712878600080, -205.0899764529922038 ) ) ;
#1231=CARTESIAN_POINT ( 'NONE',  ( -44.67521729214921322, -296.9037517187510957, -346.0457820422524264 ) ) ;
#1232=CARTESIAN_POINT ( 'NONE',  ( -41.60269001370426878, -292.4895289931519642, -197.3740484606091172 ) ) ;
#1233=CARTESIAN_POINT ( 'NONE',  ( -99.38399009088003311, -274.0962103606051414, -225.0670462314396048 ) ) ;
#1234=CARTESIAN_POINT ( 'NONE',  ( 12.47787929332878498, -287.0257133110566201, -324.4603671640349489 ) ) ;
#1235=CARTESIAN_POINT ( 'NONE',  ( -66.19667825136785666, -274.3356543446176943, -199.0679154175945484 ) ) ;
#1236=CARTESIAN_POINT ( 'NONE',  ( -69.25945243168244758, -297.7867702038719244, -204.7085697271741083 ) ) ;
#1239=CARTESIAN_POINT ( 'NONE',  ( -95.72076983864123179, -281.1291109105193868, -222.3701828786022077 ) ) ;
#1241=CARTESIAN_POINT ( 'NONE',  ( -94.18890406394115189, -280.2842494856001849, -224.0726585210119310 ) ) ;
#1242=CARTESIAN_POINT ( 'NONE',  ( -110.8414872854830833, -280.0671331399246924, -289.6931427410897868 ) ) ;
#1243=CARTESIAN_POINT ( 'NONE',  ( -21.76881556398774720, -272.7352590174109537, -198.3320056955437281 ) ) ;
#1246=CARTESIAN_POINT ( 'NONE',  ( -79.05660610622193474, -279.6384712174848346, -210.4539679608586482 ) ) ;
#1247=CARTESIAN_POINT ( 'NONE',  ( 22.62589851958319898, -275.7098621028263778, -222.2981301742025266 ) ) ;
#1248=CARTESIAN_POINT ( 'NONE',  ( 36.76375887619934701, -277.7047962690376721, -282.2368622495716863 ) ) ;
#1249=CARTESIAN_POINT ( 'NONE',  ( -86.72829848125643082, -276.2976626089749175, -328.7361955000521334 ) ) ;
#1252=CARTESIAN_POINT ( 'NONE',  ( -24.78235124978375481, -284.8727238771388102, -344.7152890780492953 ) ) ;
#1253=CARTESIAN_POINT ( 'NONE',  ( -88.03512400441982777, -290.5182726999854594, -217.5390677845554990 ) ) ;
#1254=EDGE_CURVE ( 'NONE', #75524, #47701, #79849, .T. ) ;
#1255=CARTESIAN_POINT ( 'NONE',  ( 14.18474048092872941, -286.1018353062679580, -213.2078114396948081 ) ) ;
#1256=CARTESIAN_POINT ( 'NONE',  ( -51.22971925187731301, -281.4718253673992194, -343.1120849470090661 ) ) ;
#1257=CARTESIAN_POINT ( 'NONE',  ( -53.83927818999645609, -281.8426486551438757, -342.1297666177063093 ) ) ;
#1258=CARTESIAN_POINT ( 'NONE',  ( 24.00602563254055610, -282.2005001400641504, -229.9757303430876050 ) ) ;
#1259=CARTESIAN_POINT ( 'NONE',  ( 193.6317247519612863, 279.2590634987193994, -125.8091550203929216 ) ) ;
#1260=CARTESIAN_POINT ( 'NONE',  ( -47.17353373968273900, -281.5749530826011551, -345.9241741808497181 ) ) ;
#1261=CARTESIAN_POINT ( 'NONE',  ( 31.47881924792857333, -295.1622739691200650, -240.5494296925795652 ) ) ;
#1262=CARTESIAN_POINT ( 'NONE',  ( -97.72836163025088752, -278.6311702047453878, -311.5599502583124831 ) ) ;
#1263=CARTESIAN_POINT ( 'NONE',  ( -72.77193442836117754, -287.5845644209379657, -204.0107249021278619 ) ) ;
#1265=CARTESIAN_POINT ( 'NONE',  ( -83.40815675873707846, -293.3468823295299899, -210.4019555419367862 ) ) ;
#1266=CARTESIAN_POINT ( 'NONE',  ( 28.51095958071148573, -274.0301895446212370, -306.3642975492415985 ) ) ;
#1267=CARTESIAN_POINT ( 'NONE',  ( -20.54168934993978013, -288.0390185172796009, -345.3951224932175137 ) ) ;
#1268=CARTESIAN_POINT ( 'NONE',  ( -27.98494059256432465, -290.5726294592739123, -197.1053629635317179 ) ) ;
#1269=CARTESIAN_POINT ( 'NONE',  ( -101.0184308945940046, -276.7360075648400652, -307.1582907912126643 ) ) ;
#1270=CARTESIAN_POINT ( 'NONE',  ( -103.6247257536396802, -295.1392584653447670, -236.8188105767752916 ) ) ;
#1271=CARTESIAN_POINT ( 'NONE',  ( -96.15295369221790622, -291.2525545779229219, -314.4556879514004777 ) ) ;
#1274=CARTESIAN_POINT ( 'NONE',  ( 12.92442427130810856, -292.8454988994985797, -327.8421735475841956 ) ) ;
#1275=CARTESIAN_POINT ( 'NONE',  ( -5.471426269818340238, -288.0786184467141311, -203.7834850905255166 ) ) ;
#1276=CARTESIAN_POINT ( 'NONE',  ( -112.9956661257817387, -288.8888957890508209, -262.7163230750809930 ) ) ;
#1277=CARTESIAN_POINT ( 'NONE',  ( 35.10493895194819913, -289.1464659952534930, -283.2785250020855869 ) ) ;
#1279=CARTESIAN_POINT ( 'NONE',  ( -23.74516055091860878, -289.6769305378810486, -342.2998982507519941 ) ) ;
#1282=CARTESIAN_POINT ( 'NONE',  ( -20.56832576917869915, -290.0466037300154198, -345.1594865736184943 ) ) ;
#1283=CARTESIAN_POINT ( 'NONE',  ( -58.80892421910212420, -277.7959193459898302, -198.1284031630851814 ) ) ;
#1284=CARTESIAN_POINT ( 'NONE',  ( -109.5878191296876594, -279.2231289540560510, -243.6319765235116961 ) ) ;
#1285=CARTESIAN_POINT ( 'NONE',  ( -36.74845336231327764, -279.7261383661606828, -193.3715058316192312 ) ) ;
#1286=CARTESIAN_POINT ( 'NONE',  ( -60.57463744152092033, -283.7506191264303652, -199.0503104512943935 ) ) ;
#1288=CARTESIAN_POINT ( 'NONE',  ( -36.97890755337682833, -278.1963271922607532, -196.1268006791808034 ) ) ;
#1289=CARTESIAN_POINT ( 'NONE',  ( -2.584223713412890255, -280.5922660126767596, -336.8210193129521031 ) ) ;
#1291=CARTESIAN_POINT ( 'NONE',  ( -103.0189976239582990, -276.5201896994689719, -309.3132081572083507 ) ) ;
#1292=CARTESIAN_POINT ( 'NONE',  ( -70.79946912355336508, -299.1226755514359752, -204.6866931959504257 ) ) ;
#1293=CARTESIAN_POINT ( 'NONE',  ( -109.0189814984703673, -283.1241916530127583, -297.7829623172737570 ) ) ;
#1294=CARTESIAN_POINT ( 'NONE',  ( -46.20846488888262371, -274.7396264861915824, -197.7389298480991329 ) ) ;
#1295=CARTESIAN_POINT ( 'NONE',  ( -92.75743588560285957, -274.7020742062829868, -217.7330602485023121 ) ) ;
#1296=CARTESIAN_POINT ( 'NONE',  ( 7.590064494120423610, -276.0865560307798887, -327.9861570643587356 ) ) ;
#1297=CARTESIAN_POINT ( 'NONE',  ( -34.19239939503944470, -297.0126997558913899, -345.2949725208078462 ) ) ;
#1298=CARTESIAN_POINT ( 'NONE',  ( -75.66183911080170787, -289.7155964329720632, -337.1485940005564999 ) ) ;
#1299=CARTESIAN_POINT ( 'NONE',  ( -70.57872091346399657, -277.6971733661320627, -202.5038070151277054 ) ) ;
#1300=CARTESIAN_POINT ( 'NONE',  ( -102.3024015441570782, -289.8424642856674609, -311.8005918935049294 ) ) ;
#1301=CARTESIAN_POINT ( 'NONE',  ( -61.34340426095521082, -288.4304225641278094, -339.5516277842015143 ) ) ;
#1302=CARTESIAN_POINT ( 'NONE',  ( -1.730437127795238172, -290.5239215406219273, -204.3547652704849895 ) ) ;
#1305=CARTESIAN_POINT ( 'NONE',  ( -94.15609292284101173, -289.4106324383022297, -316.2970866045370713 ) ) ;
#1307=CARTESIAN_POINT ( 'NONE',  ( -32.33377699988042053, -287.0550684935378172, -193.7468109722198619 ) ) ;
#1308=CARTESIAN_POINT ( 'NONE',  ( -92.08974858914540107, -287.6948066931273047, -226.7417163044926838 ) ) ;
#1309=CARTESIAN_POINT ( 'NONE',  ( 33.19561060100984662, -292.9993756964033764, -300.7824051068001268 ) ) ;
#1310=CARTESIAN_POINT ( 'NONE',  ( 24.71714679701682016, -283.4646391430484869, -315.1270526228138351 ) ) ;
#1311=CARTESIAN_POINT ( 'NONE',  ( -93.25373315542717023, -285.0519866982648409, -223.4266469907795454 ) ) ;
#1312=CARTESIAN_POINT ( 'NONE',  ( 15.79182080314342862, -276.1390977356639951, -219.5127464327528060 ) ) ;
#1313=CARTESIAN_POINT ( 'NONE',  ( 35.93431208748905448, -291.7558319500407720, -284.5904130878255955 ) ) ;
#1314=CARTESIAN_POINT ( 'NONE',  ( 33.89827047411661454, -274.1152497349642090, -252.6976784929620976 ) ) ;
#1315=VERTEX_POINT ( 'NONE', #89447 ) ;
#1317=CARTESIAN_POINT ( 'NONE',  ( -8.399926009726220499, -294.3503289677409498, -341.7486276080564380 ) ) ;
#1318=CARTESIAN_POINT ( 'NONE',  ( 16.04554392009131902, -288.7367144869345452, -218.4851469519760201 ) ) ;
#1319=CARTESIAN_POINT ( 'NONE',  ( -89.40857248324721240, -298.4192051437676696, -213.9816785797699197 ) ) ;
#1320=CARTESIAN_POINT ( 'NONE',  ( 18.73462360188017328, -287.5386252663560072, -223.4445128708985919 ) ) ;
#1321=CARTESIAN_POINT ( 'NONE',  ( -108.2906088729402256, -277.9845747191277496, -241.0511783668453063 ) ) ;
#1322=CARTESIAN_POINT ( 'NONE',  ( -32.01128333207816468, -295.6380054311364347, -347.0874532399008103 ) ) ;
#1323=CARTESIAN_POINT ( 'NONE',  ( 21.43170968467204318, -286.3438955711848166, -318.1935738807069924 ) ) ;
#1324=CARTESIAN_POINT ( 'NONE',  ( 34.43330939936353019, -294.2380094333950069, -298.1836322253800518 ) ) ;
#1325=CARTESIAN_POINT ( 'NONE',  ( -69.03061536482888982, -291.9568873796781645, -204.5605326833156710 ) ) ;
#1327=DIRECTION ( 'NONE',  ( 0.000000000000000000, 0.000000000000000000, -1.000000000000000000 ) ) ;
#1328=CARTESIAN_POINT ( 'NONE',  ( -54.76359932917087292, -169.9329552034514279, -360.8268486737608214 ) ) ;
#1329=CARTESIAN_POINT ( 'NONE',  ( -36.59186565410484349, -287.5815181310400135, -194.0452119181639148 ) ) ;
#1330=CARTESIAN_POINT ( 'NONE',  ( -88.52914483777347243, -281.1952119285918457, -334.4957818155094174 ) ) ;
#1332=CARTESIAN_POINT ( 'NONE',  ( -100.1609200747649027, -278.4883935519898728, -226.0095859684839468 ) ) ;
#1333=CARTESIAN_POINT ( 'NONE',  ( 20.23064365918139274, -282.8906745597048484, -222.5348204226079361 ) ) ;
#1334=CARTESIAN_POINT ( 'NONE',  ( 155.5532833854414605, 205.0543101207102552, -216.1346246433878662 ) ) ;
#1335=CARTESIAN_POINT ( 'NONE',  ( -98.85897664030493104, -283.7346967105872295, -224.9504601315421155 ) ) ;
#1336=CARTESIAN_POINT ( 'NONE',  ( 24.69633640067911173, -286.1921374569451473, -311.5255637593836013 ) ) ;
#1337=CARTESIAN_POINT ( 'NONE',  ( 23.47400430328696430, -276.8019297325512298, -225.1753284315388441 ) ) ;
#1338=CARTESIAN_POINT ( 'NONE',  ( -88.17305750314029922, -297.8096883478827408, -217.8103719788934995 ) ) ;
#1339=CARTESIAN_POINT ( 'NONE',  ( 29.93481593136025509, -292.6322940907930956, -299.9434414810605176 ) ) ;
#1340=CARTESIAN_POINT ( 'NONE',  ( -111.9889758563177651, -279.4355265076290493, -251.8382576489704547 ) ) ;
#1341=CARTESIAN_POINT ( 'NONE',  ( -21.65302150415941185, -276.8455267778230109, -341.7073272721959256 ) ) ;
#1342=CARTESIAN_POINT ( 'NONE',  ( -36.55569576436343482, -299.0030139488621899, -193.5962881258471100 ) ) ;
#1343=CARTESIAN_POINT ( 'NONE',  ( 0.8809921019165840583, -275.4753837376584897, -336.9083267520210825 ) ) ;
#1345=CARTESIAN_POINT ( 'NONE',  ( 20.43381909603769131, -274.2126301869488998, -318.2629804891827803 ) ) ;
#1346=CARTESIAN_POINT ( 'NONE',  ( -111.0190159084740742, -297.7217385083195040, -290.6159799495050038 ) ) ;
#1350=CARTESIAN_POINT ( 'NONE',  ( -81.67639484432494612, -286.5118216850802355, -211.9773795181534410 ) ) ;
#1351=CARTESIAN_POINT ( 'NONE',  ( -73.77021608239635952, -285.2887063867223105, -337.1051792772611293 ) ) ;
#1352=CARTESIAN_POINT ( 'NONE',  ( -17.13575233439146572, -285.6684329036442591, -200.0542813169454632 ) ) ;
#1353=CARTESIAN_POINT ( 'NONE',  ( -105.0130160142174276, -276.5588928881783204, -299.9346840640773166 ) ) ;
#1354=CARTESIAN_POINT ( 'NONE',  ( -111.5446812273848707, -286.4409455841696968, -268.1740940822559196 ) ) ;
#1355=CARTESIAN_POINT ( 'NONE',  ( -19.34668950920417529, -278.7676106982231090, -198.8458383650429653 ) ) ;
#1356=CARTESIAN_POINT ( 'NONE',  ( 32.39645809962343037, -276.9304153606940986, -292.9623427422388886 ) ) ;
#1358=CARTESIAN_POINT ( 'NONE',  ( 94.63317399270954411, -300.3986776538885124, -197.2442351111135963 ) ) ;
#1359=CARTESIAN_POINT ( 'NONE',  ( 29.62619520685872487, -282.8460436223892884, -308.1453017321348398 ) ) ;
#1360=CARTESIAN_POINT ( 'NONE',  ( -0.3994739115543821106, -283.0669260933392479, -337.8652953817621665 ) ) ;
#1362=EDGE_LOOP ( 'NONE', ( #389, #48035 ) ) ;
#1364=CARTESIAN_POINT ( 'NONE',  ( 36.51020841098728908, -289.1968773317620958, -253.3861411473637304 ) ) ;
#1365=CARTESIAN_POINT ( 'NONE',  ( -113.6222243893442254, -289.1547419823139649, -276.8947000431542165 ) ) ;
#1366=CARTESIAN_POINT ( 'NONE',  ( -107.0262058871500415, -295.4524755518525581, -292.8113214809180818 ) ) ;
#1368=CARTESIAN_POINT ( 'NONE',  ( -22.20572272908044553, -291.5895758068863870, -194.9131297881342277 ) ) ;
#1369=CARTESIAN_POINT ( 'NONE',  ( 10.55130591562493869, -286.8567396987317011, -326.4372153599002218 ) ) ;
#1370=CARTESIAN_POINT ( 'NONE',  ( -37.28564521386969233, -287.6261629888885523, -343.9503276333391000 ) ) ;
#1371=CARTESIAN_POINT ( 'NONE',  ( -41.35992835435267523, -287.2055487697227250, -197.0615519117667418 ) ) ;
#1372=CARTESIAN_POINT ( 'NONE',  ( -110.2374995252888681, -276.3247971859484551, -288.0559321959354975 ) ) ;
#1373=CARTESIAN_POINT ( 'NONE',  ( -29.16912478323997959, -290.9488840426138836, -344.9666562665581750 ) ) ;
#1374=CARTESIAN_POINT ( 'NONE',  ( -37.52335318451943635, -287.0542291568665405, -345.5403296610969051 ) ) ;
#1375=CARTESIAN_POINT ( 'NONE',  ( -110.4639598478855333, -285.5578378642339317, -265.4613663405748412 ) ) ;
#1376=CARTESIAN_POINT ( 'NONE',  ( -110.1399438166561708, -292.3117252194971911, -289.1326928361215778 ) ) ;
#1377=CARTESIAN_POINT ( 'NONE',  ( 82.13662659784047548, -300.5150969315919838, -193.6047415040562498 ) ) ;
#1379=CARTESIAN_POINT ( 'NONE',  ( -112.1790098971907668, -298.6063709220446754, -259.8417975139061014 ) ) ;
#1380=CARTESIAN_POINT ( 'NONE',  ( -9.175753616059115103, -279.6272733076894497, -202.8386684985784143 ) ) ;
#1381=CARTESIAN_POINT ( 'NONE',  ( 36.02688869273971051, -279.3514737429551928, -254.7418426853482742 ) ) ;
#1382=CARTESIAN_POINT ( 'NONE',  ( 39.06670442241018293, -292.6414538926898672, -261.7541836717572323 ) ) ;
#1383=CARTESIAN_POINT ( 'NONE',  ( -94.54750324048427501, -271.4483917101229054, -223.3788747945172588 ) ) ;
#1384=CARTESIAN_POINT ( 'NONE',  ( 10.57262087529013073, -274.4640251165277505, -327.3306891391998192 ) ) ;
#1385=CARTESIAN_POINT ( 'NONE',  ( -108.7744014947930111, -297.6402048737558061, -287.6945511815222289 ) ) ;
#1387=CARTESIAN_POINT ( 'NONE',  ( -91.98409470737627203, -294.0590528655447997, -323.1643634114109318 ) ) ;
#1388=CARTESIAN_POINT ( 'NONE',  ( 16.60333062456019704, -295.6910400073747383, -320.4141755769032329 ) ) ;
#1390=CARTESIAN_POINT ( 'NONE',  ( -69.78650493502040320, -296.2935837162376629, -335.9350180386305169 ) ) ;
#1392=CARTESIAN_POINT ( 'NONE',  ( -66.52821591130842194, -283.6919026314164967, -200.8877122727009237 ) ) ;
#1393=CARTESIAN_POINT ( 'NONE',  ( -108.8847233520359197, -296.3598946323040764, -284.9352898441010211 ) ) ;
#1394=CARTESIAN_POINT ( 'NONE',  ( -114.3407659224605766, -284.5568958099508450, -269.9818202197658934 ) ) ;
#1395=CARTESIAN_POINT ( 'NONE',  ( 37.84780553902246680, -283.5740164944031676, -278.3416710924523159 ) ) ;
#1396=CARTESIAN_POINT ( 'NONE',  ( -65.86558042004320157, -285.3557758935428978, -198.8477890740071246 ) ) ;
#1397=CARTESIAN_POINT ( 'NONE',  ( 35.74574881223696110, -291.3444308111306214, -254.2315161905954142 ) ) ;
#1398=CARTESIAN_POINT ( 'NONE',  ( -112.0780845840028945, -277.6733258455329292, -288.5211455284123758 ) ) ;
#1399=CARTESIAN_POINT ( 'NONE',  ( -37.37352853689063181, -280.5523547857346784, -345.3611179825600175 ) ) ;
#1401=CARTESIAN_POINT ( 'NONE',  ( 32.65688275607818269, -286.0555277732573813, -248.2434858962869839 ) ) ;
#1402=CARTESIAN_POINT ( 'NONE',  ( -46.00456630510468869, -288.0797573760335695, -346.6140794719176483 ) ) ;
#1404=CARTESIAN_POINT ( 'NONE',  ( -104.4493723474346751, -279.5009052287889517, -306.9010498480661226 ) ) ;
#1405=CARTESIAN_POINT ( 'NONE',  ( 18.29781725470346032, -292.2790196284022386, -321.2568800984311679 ) ) ;
#1406=CARTESIAN_POINT ( 'NONE',  ( 29.33203249001316593, -281.6212203201883426, -300.2627754168768206 ) ) ;
#1407=CARTESIAN_POINT ( 'NONE',  ( 37.78439455871049546, -293.9307334786635124, -287.3046512182173160 ) ) ;
#1408=CARTESIAN_POINT ( 'NONE',  ( 25.17985865037724125, -285.0616745523148552, -227.9072402999705389 ) ) ;
#1409=CARTESIAN_POINT ( 'NONE',  ( -47.86405180145010974, -281.9186281289387352, -196.0504666327389600 ) ) ;
#1411=CARTESIAN_POINT ( 'NONE',  ( -80.30245814932901283, -294.7091538289109849, -329.6720083629043643 ) ) ;
#1412=CARTESIAN_POINT ( 'NONE',  ( -108.3611493555414995, -270.8699978521538583, -245.7386433506795527 ) ) ;
#1415=CARTESIAN_POINT ( 'NONE',  ( 33.80659575920257254, -283.8267560256765023, -293.1076588587019387 ) ) ;
#1416=CARTESIAN_POINT ( 'NONE',  ( -61.03904947665057534, -294.8757426141323776, -339.5264176675144085 ) ) ;
#1418=CARTESIAN_POINT ( 'NONE',  ( -106.6662871844225293, -281.6237833571634610, -303.7098442033569086 ) ) ;
#1419=CARTESIAN_POINT ( 'NONE',  ( -71.32217281691825406, -272.8120242918620875, -201.4446011151220830 ) ) ;
#1422=CARTESIAN_POINT ( 'NONE',  ( -98.11185000843182991, -289.8237282426162551, -310.8312352110697248 ) ) ;
#1423=CARTESIAN_POINT ( 'NONE',  ( -89.98227290016242819, -280.8123861596716893, -218.7167137960210539 ) ) ;
#1424=CARTESIAN_POINT ( 'NONE',  ( -16.43331552015228425, -275.9268990689354837, -199.5315708164286832 ) ) ;
#1425=CARTESIAN_POINT ( 'NONE',  ( -19.09005687647491101, -284.4213199808800141, -344.3973838385429644 ) ) ;
#1426=CARTESIAN_POINT ( 'NONE',  ( -64.95132935486626025, -278.4781689442403376, -202.3549500325787278 ) ) ;
#1427=CARTESIAN_POINT ( 'NONE',  ( -51.63783561217644547, -279.2352042517546806, -343.9859857652226651 ) ) ;
#1429=CARTESIAN_POINT ( 'NONE',  ( -90.16131540396499133, -273.1635997788909549, -214.2607405942027867 ) ) ;
#1430=CARTESIAN_POINT ( 'NONE',  ( -102.3937442989139015, -292.9587663097002519, -234.0675382806387574 ) ) ;
#1433=CARTESIAN_POINT ( 'NONE',  ( -33.52120502682937797, -293.1441615915895795, -346.0424438696508105 ) ) ;
#1434=CARTESIAN_POINT ( 'NONE',  ( 19.90763343179916589, -274.4194142080881988, -224.9483417611401421 ) ) ;
#1435=CARTESIAN_POINT ( 'NONE',  ( -58.76276249475572655, -293.3000997861807377, -197.1228367477258132 ) ) ;
#1436=CARTESIAN_POINT ( 'NONE',  ( 35.77081079830085031, -277.8376638359845288, -253.6410175316879361 ) ) ;
#1437=CARTESIAN_POINT ( 'NONE',  ( -37.80809119427475196, -293.2515017321359778, -193.7596088598672850 ) ) ;
#1438=CARTESIAN_POINT ( 'NONE',  ( 36.57399071147558089, -289.7037128773318386, -282.1262348526219057 ) ) ;
#1439=CARTESIAN_POINT ( 'NONE',  ( 34.26340533266121469, -273.8333595633521327, -292.1480107064741674 ) ) ;
#1440=CARTESIAN_POINT ( 'NONE',  ( 28.04306295079809885, -277.9498730916036493, -306.0518975365675374 ) ) ;
#1441=CARTESIAN_POINT ( 'NONE',  ( -3.707476465593006143, -292.6847075651662067, -336.7836217841268081 ) ) ;
#1442=CARTESIAN_POINT ( 'NONE',  ( -103.7229564553331613, -280.8932924034027110, -233.8394218753010989 ) ) ;
#1444=CARTESIAN_POINT ( 'NONE',  ( -26.74390006549232979, -282.5804926980131881, -342.6604363933534501 ) ) ;
#1445=CARTESIAN_POINT ( 'NONE',  ( -53.70797439407711948, -280.9266823302423290, -195.3825539801070192 ) ) ;
#1446=CARTESIAN_POINT ( 'NONE',  ( -24.61474080773121997, -281.6882686554803286, -345.9532429516009984 ) ) ;
#1447=CARTESIAN_POINT ( 'NONE',  ( -95.02603804343112870, -278.8058644561330652, -321.0102776263897795 ) ) ;
#1448=CARTESIAN_POINT ( 'NONE',  ( 23.91164583182238701, -276.4616907791411791, -224.8557846361411521 ) ) ;
#1449=CARTESIAN_POINT ( 'NONE',  ( 30.89617123739170168, -289.8376638359844719, -254.7536222014695397 ) ) ;
#1452=CARTESIAN_POINT ( 'NONE',  ( -109.3874940036984640, -298.8206270639723243, -249.5187516343233654 ) ) ;
#1453=CARTESIAN_POINT ( 'NONE',  ( -25.37210858833041982, -293.2878451266919342, -197.9840818391974722 ) ) ;
#1454=CARTESIAN_POINT ( 'NONE',  ( -108.6962292960956091, -276.2863250136849729, -292.4519222031888148 ) ) ;
#1455=CARTESIAN_POINT ( 'NONE',  ( -15.22547718514172388, -290.5299158293701680, -343.1130917346178535 ) ) ;
#1456=CARTESIAN_POINT ( 'NONE',  ( -66.59726230471117958, -291.0070993842258531, -203.3685456317933244 ) ) ;
#1457=CARTESIAN_POINT ( 'NONE',  ( 3.142418115635885911, -288.0318454059959095, -335.8496251866239390 ) ) ;
#1459=CARTESIAN_POINT ( 'NONE',  ( -111.1911077235709087, -282.9450498158478808, -270.8949704174044086 ) ) ;
#1460=CARTESIAN_POINT ( 'NONE',  ( -110.6349106926464145, -292.2586127777328784, -282.2295021675640783 ) ) ;
#1461=CARTESIAN_POINT ( 'NONE',  ( -108.4350998182151926, -282.7775506637423177, -289.8107735325176009 ) ) ;
#1462=CARTESIAN_POINT ( 'NONE',  ( -9.073033251643639829, -281.7449377755394835, -202.5221472374239511 ) ) ;
#1464=CARTESIAN_POINT ( 'NONE',  ( -97.96638673433362499, -290.8625750643865899, -317.4511125449042765 ) ) ;
#1465=CARTESIAN_POINT ( 'NONE',  ( -89.52191759520569292, -279.7847770721391498, -219.1502558904300599 ) ) ;
#1466=CARTESIAN_POINT ( 'NONE',  ( -44.84281161810447713, -290.7542629961829448, -194.0736863607303917 ) ) ;
#1467=CARTESIAN_POINT ( 'NONE',  ( 21.95902065947467818, -287.6970775699344358, -221.4982145150968620 ) ) ;
#1468=CARTESIAN_POINT ( 'NONE',  ( 7.903391843717010090, -288.9450214563344730, -332.6554997890902996 ) ) ;
#1469=CARTESIAN_POINT ( 'NONE',  ( -72.37587749378877788, -285.7415138044681271, -206.3031160916555677 ) ) ;
#1472=CARTESIAN_POINT ( 'NONE',  ( 19.43705777708717264, -294.7219535435830835, -220.1770140457471427 ) ) ;
#1473=CARTESIAN_POINT ( 'NONE',  ( -22.21155743937168126, -293.5470792457638822, -345.3569648920415602 ) ) ;
#1474=CARTESIAN_POINT ( 'NONE',  ( -61.87991936387788883, -276.4376941382475366, -339.4170950671252740 ) ) ;
#1475=CARTESIAN_POINT ( 'NONE',  ( -54.56426064149214028, -297.1850267285084897, -195.4164971240218449 ) ) ;
#1477=CARTESIAN_POINT ( 'NONE',  ( 19.35423114739423056, -292.6934918920479731, -317.4384918592071472 ) ) ;
#1478=CARTESIAN_POINT ( 'NONE',  ( -111.2224919485975789, -294.8496100106004292, -265.9336343442270731 ) ) ;
#1479=CARTESIAN_POINT ( 'NONE',  ( -79.77269421180812969, -292.6695535082092761, -210.4094046147227175 ) ) ;
#1480=CARTESIAN_POINT ( 'NONE',  ( 12.57537448609780029, -295.4166087703552535, -324.1197342669860291 ) ) ;
#1483=CARTESIAN_POINT ( 'NONE',  ( 24.97718621167626196, -292.1192734698619802, -312.3894992523332803 ) ) ;
#1484=AXIS2_PLACEMENT_3D ( 'NONE', #68828, #19100, #3957 ) ;
#1485=CARTESIAN_POINT ( 'NONE',  ( -100.9186871615504373, -299.0880780845530467, -230.4781179084328642 ) ) ;
#1486=CARTESIAN_POINT ( 'NONE',  ( -107.6244744988845810, -291.7653974983800254, -249.7316160731506045 ) ) ;
#1487=CARTESIAN_POINT ( 'NONE',  ( 8.244676534088640096, -294.7421266707629570, -327.4696829607519248 ) ) ;
#1488=CARTESIAN_POINT ( 'NONE',  ( -96.42336048847371899, -281.1715587650895145, -223.5875761371995054 ) ) ;
#1489=CARTESIAN_POINT ( 'NONE',  ( -95.51983067280377782, -277.9116797784892583, -220.6559596598636404 ) ) ;
#1490=CARTESIAN_POINT ( 'NONE',  ( -111.7175489734729439, -272.1479081000331917, -250.6242070340624650 ) ) ;
#1491=CARTESIAN_POINT ( 'NONE',  ( 35.04479773637792306, -279.8573300613501260, -287.7792932032427302 ) ) ;
#1492=CARTESIAN_POINT ( 'NONE',  ( -94.34960562910202952, -277.6443057176829257, -219.7988877434916333 ) ) ;
#1493=CARTESIAN_POINT ( 'NONE',  ( -107.8767749087758290, -276.8900631826272161, -244.2334650969371808 ) ) ;
#1494=CARTESIAN_POINT ( 'NONE',  ( -33.76528826327452038, -296.7826661299722559, -196.8687839923029230 ) ) ;
#1495=CARTESIAN_POINT ( 'NONE',  ( -102.6196903255425923, -275.0456344671761144, -233.3280175503710439 ) ) ;
#1497=CARTESIAN_POINT ( 'NONE',  ( -110.3352241451626128, -288.3323161655783906, -289.1305061886560566 ) ) ;
#1498=CARTESIAN_POINT ( 'NONE',  ( -109.8655511909556992, -290.2238299034394231, -296.3898506772237624 ) ) ;
#1499=CARTESIAN_POINT ( 'NONE',  ( 10.59640682969090797, -276.7123369522162761, -212.3973327032843486 ) ) ;
#1500=CARTESIAN_POINT ( 'NONE',  ( -102.4414457841392334, -271.0499318755020113, -233.0139747473175476 ) ) ;
#1501=CARTESIAN_POINT ( 'NONE',  ( -61.19128421136908003, -282.5511546251398158, -343.4602108481794858 ) ) ;
#1503=CARTESIAN_POINT ( 'NONE',  ( -55.75508799387365855, -281.2888926331569905, -343.1185365373967215 ) ) ;
#1504=DIRECTION ( 'NONE',  ( 0.000000000000000000, 0.000000000000000000, 1.000000000000000000 ) ) ;
#1505=CARTESIAN_POINT ( 'NONE',  ( 34.87661588333293139, -292.1742611994909566, -257.1898032103383684 ) ) ;
#1506=CARTESIAN_POINT ( 'NONE',  ( -80.00003502251276188, -283.6081244029235791, -209.5433377442685696 ) ) ;
#1509=CARTESIAN_POINT ( 'NONE',  ( -0.2458855626439184761, -290.5452906424620210, -205.1626475860752237 ) ) ;
#1510=CARTESIAN_POINT ( 'NONE',  ( -68.35526443095929494, -279.0666212601479970, -337.3421645641082023 ) ) ;
#1511=CARTESIAN_POINT ( 'NONE',  ( 0.6846499462318222928, -283.7619552028866110, -336.8744341544945087 ) ) ;
#1512=CARTESIAN_POINT ( 'NONE',  ( -80.40917117863796193, -271.5538468486288934, -208.2130509116692281 ) ) ;
#1513=CARTESIAN_POINT ( 'NONE',  ( -99.60931826203945150, -285.0783202633334668, -232.1630526575822842 ) ) ;
#1514=CARTESIAN_POINT ( 'NONE',  ( 29.69846770327152896, -277.3831657951517400, -300.7089484258265202 ) ) ;
#1515=CARTESIAN_POINT ( 'NONE',  ( -11.18678636406967186, -277.5051935538521661, -338.6877029478237091 ) ) ;
#1516=CARTESIAN_POINT ( 'NONE',  ( -102.6622816111977556, -286.0600908051282545, -307.3203115391984852 ) ) ;
#1519=CARTESIAN_POINT ( 'NONE',  ( -56.07233749544652568, -295.1202883827519372, -345.0482201374624083 ) ) ;
#1520=CARTESIAN_POINT ( 'NONE',  ( 34.24027624111162282, -289.2576488976930023, -249.1532017050213881 ) ) ;
#1521=PLANE ( 'NONE',  #44283 ) ;
#1522=CARTESIAN_POINT ( 'NONE',  ( 36.60358173371529489, -290.6237833571632905, -234.7871824221999191 ) ) ;
#1523=CARTESIAN_POINT ( 'NONE',  ( -113.9014659788277157, -277.5287711341777594, -265.8783998487165263 ) ) ;
#1525=CARTESIAN_POINT ( 'NONE',  ( -37.76987282709563232, -290.4467517415907309, -194.1623182098586824 ) ) ;
#1526=CARTESIAN_POINT ( 'NONE',  ( -111.0840718524911921, -286.0647981291634210, -270.9338253024325809 ) ) ;
#1527=CARTESIAN_POINT ( 'NONE',  ( -111.1710211117971312, -280.3801643721818664, -265.1452408090502786 ) ) ;
#1528=CARTESIAN_POINT ( 'NONE',  ( 12.04888671161283931, -289.8060316138229382, -328.6635726732819194 ) ) ;
#1529=CARTESIAN_POINT ( 'NONE',  ( 17.29998704130776233, -284.2728057879130006, -321.8100623489077066 ) ) ;
#1530=CARTESIAN_POINT ( 'NONE',  ( -9.209842786283447325, -276.8610115028255905, -342.0381617762970450 ) ) ;
#1531=CARTESIAN_POINT ( 'NONE',  ( -39.18421180120234482, -296.0490574145894129, -195.7263683417058360 ) ) ;
#1532=CARTESIAN_POINT ( 'NONE',  ( -41.00627162774281231, -279.8405853337705480, -193.4351737076655979 ) ) ;
#1534=CARTESIAN_POINT ( 'NONE',  ( -108.8493213664828261, -298.7406335615847865, -249.6735781582797529 ) ) ;
#1538=CARTESIAN_POINT ( 'NONE',  ( -73.44339699170770075, -271.8202371963305950, -203.4397772358568091 ) ) ;
#1540=CARTESIAN_POINT ( 'NONE',  ( -110.0266555542237370, -278.1638359122140969, -262.4681452224736518 ) ) ;
#1541=CARTESIAN_POINT ( 'NONE',  ( 5.661122632621188977, -277.6885939791913529, -333.7548554677638322 ) ) ;
#1543=CARTESIAN_POINT ( 'NONE',  ( -55.65768918071592708, -282.3410986941567558, -344.9087185965823892 ) ) ;
#1544=CARTESIAN_POINT ( 'NONE',  ( 23.59678886155491995, -289.8895293847145922, -312.3891160001019784 ) ) ;
#1545=CARTESIAN_POINT ( 'NONE',  ( -37.27381386635783400, -299.5731044153225184, -194.0536722989971850 ) ) ;
#1546=CARTESIAN_POINT ( 'NONE',  ( -43.27439573798378092, -299.1840176812871164, -193.9353343587565348 ) ) ;
#1547=CARTESIAN_POINT ( 'NONE',  ( 27.81869143408052381, -295.0596889637145637, -233.4565744346762131 ) ) ;
#1548=CARTESIAN_POINT ( 'NONE',  ( 37.52205576741398119, -279.5288648170840133, -268.5643515860454613 ) ) ;
#1549=CARTESIAN_POINT ( 'NONE',  ( 14.95337341170095691, -284.2284178440503410, -323.4105009922290037 ) ) ;
#1550=CARTESIAN_POINT ( 'NONE',  ( -24.28447781559408725, -272.2396343130468495, -196.8144476749051250 ) ) ;
#1551=CARTESIAN_POINT ( 'NONE',  ( -95.64491491427668279, -285.4844500834294081, -319.4442754478668576 ) ) ;
#1552=CARTESIAN_POINT ( 'NONE',  ( -31.86191381937559441, -287.9018474164876693, -343.5159773154330196 ) ) ;
#1553=CARTESIAN_POINT ( 'NONE',  ( 140.5102961050414763, 179.4691865189072359, -241.1533972869285947 ) ) ;
#1555=CARTESIAN_POINT ( 'NONE',  ( 37.24578009612667273, -286.3367520131498623, -287.0133803577105596 ) ) ;
#1556=CARTESIAN_POINT ( 'NONE',  ( 30.50325596076029555, -287.5816946940914818, -297.5002385342463640 ) ) ;
#1558=CARTESIAN_POINT ( 'NONE',  ( -114.0181679633995628, -285.6722543968268724, -267.1411551968898834 ) ) ;
#1559=CARTESIAN_POINT ( 'NONE',  ( 35.04090862371136694, -275.7583618527364706, -260.7254842694100034 ) ) ;
#1560=CARTESIAN_POINT ( 'NONE',  ( 24.62835469155562507, -293.0748126654536350, -315.5629284065417437 ) ) ;
#1561=CARTESIAN_POINT ( 'NONE',  ( 11.43435798209858056, -283.0478621234250340, -329.8792427238093410 ) ) ;
#1562=CARTESIAN_POINT ( 'NONE',  ( 25.69681137297977358, -282.4989251112415900, -227.2706535599281494 ) ) ;
#1563=CARTESIAN_POINT ( 'NONE',  ( -65.24056689306723911, -283.7402202951333834, -342.1206833954711328 ) ) ;
#1564=CARTESIAN_POINT ( 'NONE',  ( 35.70842359217802198, -281.8619309966367723, -268.5788269733583320 ) ) ;
#1565=CARTESIAN_POINT ( 'NONE',  ( -109.1418805571601069, -294.0523547857346784, -270.3284710469131937 ) ) ;
#1566=CARTESIAN_POINT ( 'NONE',  ( 202.7079149121087198, 293.4844853417044988, -83.24464055084622771 ) ) ;
#1568=CARTESIAN_POINT ( 'NONE',  ( -23.97779326579380310, -278.8813625873251567, -344.0442539909758466 ) ) ;
#1569=CARTESIAN_POINT ( 'NONE',  ( -23.12974717564393501, -107.7894168028556834, -362.0842449849661762 ) ) ;
#1570=CARTESIAN_POINT ( 'NONE',  ( -110.3438963854144816, -295.8504482178817057, -274.1784481349151292 ) ) ;
#1571=CARTESIAN_POINT ( 'NONE',  ( 24.83284670563353558, -293.6620419679333622, -315.7027587331984364 ) ) ;
#1572=CARTESIAN_POINT ( 'NONE',  ( 65.57626950325040127, 46.04035155613875929, -315.5245225720349254 ) ) ;
#1574=CARTESIAN_POINT ( 'NONE',  ( -100.2551300561488716, -295.7040920794071894, -226.9733230316642505 ) ) ;
#1575=CARTESIAN_POINT ( 'NONE',  ( -83.05761992626356971, -288.0899159806922967, -328.2963843580874936 ) ) ;
#1576=CARTESIAN_POINT ( 'NONE',  ( -35.59824836245590518, -296.8904974318918448, -344.5885532932438764 ) ) ;
#1577=CARTESIAN_POINT ( 'NONE',  ( 15.37162616743650645, -288.1318320000314088, -219.1502918934397997 ) ) ;
#1579=CARTESIAN_POINT ( 'NONE',  ( 6.489514836131241360, -295.4140806042470899, -333.4468814723030050 ) ) ;
#1580=CARTESIAN_POINT ( 'NONE',  ( -57.41730933459302832, -286.2784353751287085, -200.0592000619339785 ) ) ;
#1581=CARTESIAN_POINT ( 'NONE',  ( -54.49127349994017067, -296.6314533129871052, -195.7025561786944081 ) ) ;
#1582=CARTESIAN_POINT ( 'NONE',  ( 19.28972365225641994, -293.6469338819406403, -218.4280778137662367 ) ) ;
#1583=CARTESIAN_POINT ( 'NONE',  ( 27.99678076511742475, -293.5114966892802499, -229.6352269325376483 ) ) ;
#1584=CARTESIAN_POINT ( 'NONE',  ( -104.7038899018843807, -291.0977518044177259, -242.0988807419200555 ) ) ;
#1587=CARTESIAN_POINT ( 'NONE',  ( -41.14521788562242222, -275.9249179403554990, -194.8456234185303231 ) ) ;
#1588=CARTESIAN_POINT ( 'NONE',  ( 17.81441157817552678, -273.6147887391460927, -217.1265888411712126 ) ) ;
#1590=CARTESIAN_POINT ( 'NONE',  ( -93.29355369734641101, -277.3374731295478455, -323.2477723545381991 ) ) ;
#1591=CARTESIAN_POINT ( 'NONE',  ( -69.82492212025711353, -272.0169028397427837, -204.0943789151146177 ) ) ;
#1592=CARTESIAN_POINT ( 'NONE',  ( -94.91322446383126987, -281.0648676543580677, -223.4955115175889091 ) ) ;
#1593=CARTESIAN_POINT ( 'NONE',  ( -72.25572342815260640, -275.6587097611486001, -335.8878727235614292 ) ) ;
#1594=CARTESIAN_POINT ( 'NONE',  ( -103.4898831614755039, -274.0573957815899462, -238.7597896242689899 ) ) ;
#1595=CARTESIAN_POINT ( 'NONE',  ( -38.09677444851720196, -274.9837151869672311, -197.1297154856137865 ) ) ;
#1596=CARTESIAN_POINT ( 'NONE',  ( -110.8439382731208980, -274.5590712724159062, -250.8879076638938557 ) ) ;
#1597=CARTESIAN_POINT ( 'NONE',  ( -13.55721941409112574, -272.3795423424051592, -198.8579342890237740 ) ) ;
#1598=CARTESIAN_POINT ( 'NONE',  ( -69.76182583659532099, -296.1421888589821947, -335.8807953138737616 ) ) ;
#1599=CARTESIAN_POINT ( 'NONE',  ( 14.72041401247748915, -292.8762895228433649, -322.4415078165400246 ) ) ;
#1601=CARTESIAN_POINT ( 'NONE',  ( -4.015826881889136502, -277.1167301806580099, -339.7219329248168833 ) ) ;
#1602=CARTESIAN_POINT ( 'NONE',  ( 21.47992204937843752, -275.1131098739491563, -227.1289913990223113 ) ) ;
#1603=CARTESIAN_POINT ( 'NONE',  ( -111.7435278037817454, -283.0119462341349958, -288.2398208758913825 ) ) ;
#1604=CARTESIAN_POINT ( 'NONE',  ( -104.3124203261300238, -298.1007224023215372, -304.6070781542059080 ) ) ;
#1605=CARTESIAN_POINT ( 'NONE',  ( -25.10477003004976737, -285.4092135434137845, -198.1788573615894222 ) ) ;
#1606=CARTESIAN_POINT ( 'NONE',  ( -109.3589609794314441, -282.2747094004473638, -291.9359041034900883 ) ) ;
#1607=CARTESIAN_POINT ( 'NONE',  ( -81.44086963633981213, -275.9012561383001980, -329.8021581798747093 ) ) ;
#1608=CARTESIAN_POINT ( 'NONE',  ( -43.27252726397514948, -275.7032369514942047, -343.7109660178809918 ) ) ;
#1610=CARTESIAN_POINT ( 'NONE',  ( -51.28233074770404443, -281.8742238388606438, -196.6158302983829742 ) ) ;
#1611=CARTESIAN_POINT ( 'NONE',  ( 35.50211883959628523, -276.8805763525704720, -279.7620530667037997 ) ) ;
#1613=CARTESIAN_POINT ( 'NONE',  ( 24.68765769267331578, -273.3593948587888462, -226.0804652099130010 ) ) ;
#1615=CARTESIAN_POINT ( 'NONE',  ( -72.92088819288660773, -281.5820908632840656, -204.1336082957760425 ) ) ;
#1617=CARTESIAN_POINT ( 'NONE',  ( 21.84831040855851469, -288.8315702692190143, -223.3739541679873355 ) ) ;
#1619=CARTESIAN_POINT ( 'NONE',  ( -83.46247577153260977, -289.4201316962644910, -211.1532311690369852 ) ) ;
#1621=CARTESIAN_POINT ( 'NONE',  ( -60.62740868408015871, -296.5383017693818033, -200.7020011217740603 ) ) ;
#1622=CARTESIAN_POINT ( 'NONE',  ( -65.77857512665582362, -289.8157886128017253, -201.7747179894851115 ) ) ;
#1623=CARTESIAN_POINT ( 'NONE',  ( 202.9738562182569694, 291.4636489450776367, -54.00000000000002132 ) ) ;
#1625=CARTESIAN_POINT ( 'NONE',  ( 14.12169607694052154, -286.8252731300303822, -326.7729787424775054 ) ) ;
#1626=CARTESIAN_POINT ( 'NONE',  ( -61.78063094932833366, -284.9751209561533756, -340.0509784335445715 ) ) ;
#1627=CARTESIAN_POINT ( 'NONE',  ( -113.1983268329517500, -282.7253018832102498, -275.6249542651085562 ) ) ;
#1628=CARTESIAN_POINT ( 'NONE',  ( -106.5712913338532104, -290.8597095495214830, -247.2037497926789058 ) ) ;
#1629=CARTESIAN_POINT ( 'NONE',  ( 5.249533110438283856, -282.0664097247295103, -210.3497709975815440 ) ) ;
#1630=CARTESIAN_POINT ( 'NONE',  ( 21.94878897923050687, -282.9535193080128579, -313.2456052752808091 ) ) ;
#1632=CARTESIAN_POINT ( 'NONE',  ( -45.81522711214778099, -291.1388278857802447, -345.2903830732265646 ) ) ;
#1633=CARTESIAN_POINT ( 'NONE',  ( -35.83027923402509884, -298.2372649447141839, -193.3610765279775308 ) ) ;
#1635=CARTESIAN_POINT ( 'NONE',  ( 33.70987938463910893, -285.9646333182316198, -296.2228784914229323 ) ) ;
#1636=CARTESIAN_POINT ( 'NONE',  ( 37.23874443599788719, -275.7918163529477056, -289.5120262801918329 ) ) ;
#1637=CARTESIAN_POINT ( 'NONE',  ( -33.44728051850636774, -294.0812828094680640, -195.8052002624553722 ) ) ;
#1639=CARTESIAN_POINT ( 'NONE',  ( -20.25526795762937127, -288.7662352645560304, -195.3538533559490702 ) ) ;
#1640=CARTESIAN_POINT ( 'NONE',  ( -104.7137483946727485, -276.1118192998647487, -303.8105025117007472 ) ) ;
#1642=CARTESIAN_POINT ( 'NONE',  ( -51.63041121882034901, -296.2723257764641289, -195.4590116835833271 ) ) ;
#1643=CARTESIAN_POINT ( 'NONE',  ( 23.88339583151003254, -274.3480442087875986, -230.4189060645270217 ) ) ;
#1644=CARTESIAN_POINT ( 'NONE',  ( -86.40492894914859789, -292.8767248358395818, -215.3059888203697483 ) ) ;
#1645=CARTESIAN_POINT ( 'NONE',  ( -102.6247317423333527, -291.9440526826926430, -237.0594543679127071 ) ) ;
#1646=CARTESIAN_POINT ( 'NONE',  ( -108.3332381675128033, -286.5875715375530035, -249.2505357775856112 ) ) ;
#1647=CARTESIAN_POINT ( 'NONE',  ( 18.96906400359628719, -294.2692731210215129, -218.7112957561428175 ) ) ;
#1648=CARTESIAN_POINT ( 'NONE',  ( 23.57236081994135191, -294.2462215614904153, -224.0494428861379674 ) ) ;
#1649=CARTESIAN_POINT ( 'NONE',  ( -28.89808635804783421, -294.7755900316942643, -342.9221680128125058 ) ) ;
#1650=CARTESIAN_POINT ( 'NONE',  ( 30.03535396789157730, -289.9866415594360092, -303.3055139700287555 ) ) ;
#1651=CARTESIAN_POINT ( 'NONE',  ( -38.73041907186327393, -283.2357985498580888, -347.3485940044810150 ) ) ;
#1652=CARTESIAN_POINT ( 'NONE',  ( -56.99122451320729965, -295.8806285197832153, -197.3465436105504409 ) ) ;
#1653=CARTESIAN_POINT ( 'NONE',  ( -98.04573195976770705, -283.7525300390229290, -317.7322117414312288 ) ) ;
#1654=CARTESIAN_POINT ( 'NONE',  ( -21.27495461195972126, -278.8251003981005738, -343.3094607102461282 ) ) ;
#1656=CARTESIAN_POINT ( 'NONE',  ( -68.93200677907188378, -284.4221688895109423, -204.0963455160231206 ) ) ;
#1657=CARTESIAN_POINT ( 'NONE',  ( 34.46303846749501787, -285.8316026620146886, -292.0639301913859640 ) ) ;
#1658=CARTESIAN_POINT ( 'NONE',  ( -105.0607483084268523, -277.1372776232107071, -236.2673513917142714 ) ) ;
#1659=CARTESIAN_POINT ( 'NONE',  ( 5.045406874201050940, -57.93311274753654061, -355.0152878038887820 ) ) ;
#1660=CARTESIAN_POINT ( 'NONE',  ( -110.3706500880485493, -284.0885611170499487, -268.1791672015494328 ) ) ;
#1661=CARTESIAN_POINT ( 'NONE',  ( 23.94669089585513788, -283.3719839339678401, -316.3148103849359813 ) ) ;
#1662=CARTESIAN_POINT ( 'NONE',  ( -54.46084228448783904, -288.3255161109215692, -345.2471763931627606 ) ) ;
#1663=CARTESIAN_POINT ( 'NONE',  ( -101.4131643431225314, -279.6042918162672777, -311.7040340098704974 ) ) ;
#1664=CARTESIAN_POINT ( 'NONE',  ( -4.193266073220160095, -277.9394237644120267, -339.3282602488646944 ) ) ;
#1665=CARTESIAN_POINT ( 'NONE',  ( -93.93918323399981318, -279.0380998051352890, -224.2555336070021212 ) ) ;
#1666=CARTESIAN_POINT ( 'NONE',  ( 16.61875949127060892, -276.8037087073536782, -218.7100151731984852 ) ) ;
#1667=CARTESIAN_POINT ( 'NONE',  ( 33.58617426899444069, -285.2428112634257218, -246.5018418112450433 ) ) ;
#1668=CARTESIAN_POINT ( 'NONE',  ( -100.0109376011833859, -291.5737769913471880, -313.7086333703326204 ) ) ;
#1669=CARTESIAN_POINT ( 'NONE',  ( -28.87386692168243840, -293.8627457906940776, -343.2307640320604492 ) ) ;
#1672=CARTESIAN_POINT ( 'NONE',  ( 8.238055427622166249, -294.0756715581831031, -327.4749674202749361 ) ) ;
#1673=CARTESIAN_POINT ( 'NONE',  ( -92.59894787587302289, -292.3634276051635652, -217.1053951106169677 ) ) ;
#1674=CARTESIAN_POINT ( 'NONE',  ( 27.86857600094925047, -281.7542677208724058, -237.2108550677822052 ) ) ;
#1675=CARTESIAN_POINT ( 'NONE',  ( -99.36982232666682080, -272.2140105371391883, -225.0476431559881405 ) ) ;
#1676=CARTESIAN_POINT ( 'NONE',  ( 38.01006813017163921, -288.3957084094379297, -285.7046445438832052 ) ) ;
#1677=CARTESIAN_POINT ( 'NONE',  ( -71.89317434194919088, -289.8296844647853732, -339.1502153838598019 ) ) ;
#1678=CARTESIAN_POINT ( 'NONE',  ( 6.936376980029636208, -287.0068658301630080, -212.2322763371211352 ) ) ;
#1679=CARTESIAN_POINT ( 'NONE',  ( 193.6317248235833404, 279.2590636267979107, -125.8091547552216696 ) ) ;
#1680=CARTESIAN_POINT ( 'NONE',  ( -40.95723928608203579, -138.9634190178281017, -362.8174797514035959 ) ) ;
#1681=CARTESIAN_POINT ( 'NONE',  ( -110.1558835859493968, -268.3047593149524914, -295.2634325463859000 ) ) ;
#1683=CARTESIAN_POINT ( 'NONE',  ( -68.11462822946306517, -276.6640491675283329, -336.7498066479569729 ) ) ;
#1684=CARTESIAN_POINT ( 'NONE',  ( -109.0700602599650608, -277.2735774419044787, -285.5027304255098670 ) ) ;
#1685=CARTESIAN_POINT ( 'NONE',  ( -104.2090589165651693, -272.7155564601540050, -232.1162379136689538 ) ) ;
#1686=CARTESIAN_POINT ( 'NONE',  ( 140.1414760274805076, 178.0338941539027928, -239.0129668939350722 ) ) ;
#1687=CARTESIAN_POINT ( 'NONE',  ( -72.62822590452525162, -276.1942376163574977, -338.2591537605787835 ) ) ;
#1688=CARTESIAN_POINT ( 'NONE',  ( -63.89086097342256210, -297.1538220072495164, -341.5588431689091635 ) ) ;
#1689=CARTESIAN_POINT ( 'NONE',  ( -99.76743922069182702, -291.5668651502261923, -232.4004075003451248 ) ) ;
#1690=CARTESIAN_POINT ( 'NONE',  ( -40.44399816664863323, -298.8170463662104339, -193.5332289811452142 ) ) ;
#1691=CARTESIAN_POINT ( 'NONE',  ( 10.42314873493027605, -287.0616546680848842, -326.2832302609623980 ) ) ;
#1692=CARTESIAN_POINT ( 'NONE',  ( -70.09590052288301365, -274.2833510363454934, -200.7731998446884063 ) ) ;
#1693=CARTESIAN_POINT ( 'NONE',  ( -105.8065692134149742, -297.0583119299714099, -244.8862325304627632 ) ) ;
#1696=CARTESIAN_POINT ( 'NONE',  ( -70.62278491564876504, -281.5368598035303194, -202.5254076392495506 ) ) ;
#1697=CARTESIAN_POINT ( 'NONE',  ( -99.73802623321135741, -280.1613682758161303, -231.7814645895975048 ) ) ;
#1698=CARTESIAN_POINT ( 'NONE',  ( -102.5536271241169999, -280.8288154844870519, -231.2539062438021062 ) ) ;
#1699=CARTESIAN_POINT ( 'NONE',  ( -69.77886387602367790, -272.0968963081243146, -204.1905946158020697 ) ) ;
#1702=CARTESIAN_POINT ( 'NONE',  ( 27.78043308788700472, -281.2696125430865663, -237.2625616980432994 ) ) ;
#1703=CARTESIAN_POINT ( 'NONE',  ( 21.61332023554981419, -277.0195259890290345, -319.6405700392683684 ) ) ;
#1704=CARTESIAN_POINT ( 'NONE',  ( 37.63089621855161226, -277.5262850220284463, -268.3336952890500129 ) ) ;
#1705=CARTESIAN_POINT ( 'NONE',  ( -73.83156038324176507, -276.1016415619488953, -337.5109186801022929 ) ) ;
#1708=CARTESIAN_POINT ( 'NONE',  ( 14.63759705836963931, -284.3045538116586499, -324.9189722741356832 ) ) ;
#1709=CARTESIAN_POINT ( 'NONE',  ( -41.59201825942352571, -291.1945583554368113, -197.2732493876959268 ) ) ;
#1710=CARTESIAN_POINT ( 'NONE',  ( -57.72092388568977128, -285.1444226616906690, -196.1573414579531232 ) ) ;
#1711=CARTESIAN_POINT ( 'NONE',  ( -98.38058555856424903, -282.2162676906381193, -312.3101062699920476 ) ) ;
#1712=CARTESIAN_POINT ( 'NONE',  ( -93.88638208250931427, -282.4639869158099259, -317.4575494970145542 ) ) ;
#1713=CARTESIAN_POINT ( 'NONE',  ( -16.75054076332084563, -284.3998962782931130, -198.7717882874051156 ) ) ;
#1714=CARTESIAN_POINT ( 'NONE',  ( 17.34849390122006696, -282.0606634836764215, -221.4110088670058474 ) ) ;
#1715=CARTESIAN_POINT ( 'NONE',  ( -93.56973896943168256, -271.2420196192170465, -220.7283838381425483 ) ) ;
#1716=CARTESIAN_POINT ( 'NONE',  ( -19.12955568641073612, -281.2215781850163694, -344.4071103187382619 ) ) ;
#1717=CARTESIAN_POINT ( 'NONE',  ( 37.65509890419795624, -295.5154156613767782, -267.4871558678684664 ) ) ;
#1718=CARTESIAN_POINT ( 'NONE',  ( -99.25701812256976098, -278.6665012165066742, -309.3193415530338939 ) ) ;
#1719=CARTESIAN_POINT ( 'NONE',  ( -32.45174577122553217, -288.1138060289943610, -195.3408202976878556 ) ) ;
#1721=CARTESIAN_POINT ( 'NONE',  ( -1.508721186066707354, -294.4436026337680232, -203.8381007628641157 ) ) ;
#1722=CARTESIAN_POINT ( 'NONE',  ( -5.448659697826840898, -274.6324594844787725, -338.2562938210186303 ) ) ;
#1723=CARTESIAN_POINT ( 'NONE',  ( -36.09972708781004513, -288.2341572508835839, -347.2026873767308075 ) ) ;
#1724=CARTESIAN_POINT ( 'NONE',  ( 34.43051265496536928, -291.7271723914418544, -253.1259753565562391 ) ) ;
#1726=CARTESIAN_POINT ( 'NONE',  ( -87.44387726973756969, -276.4538294353628203, -324.1292807067435433 ) ) ;
#1727=CARTESIAN_POINT ( 'NONE',  ( -82.68008778736489717, -295.5650021513290540, -211.5142173663683707 ) ) ;
#1728=CARTESIAN_POINT ( 'NONE',  ( -58.81734638578565466, -290.6508741178286641, -340.6996931017167753 ) ) ;
#1729=CARTESIAN_POINT ( 'NONE',  ( 104.2209783822911646, -299.5541904835127980, -197.2595231212879128 ) ) ;
#1731=CARTESIAN_POINT ( 'NONE',  ( 12.83723111402624717, -291.2176547326198488, -212.8738793080092933 ) ) ;
#1732=CARTESIAN_POINT ( 'NONE',  ( -10.47754207642720381, -288.0086995450054133, -201.6105746577587468 ) ) ;
#1733=CARTESIAN_POINT ( 'NONE',  ( -109.4619355597749433, -289.0991326456193065, -246.2665912077229109 ) ) ;
#1734=CARTESIAN_POINT ( 'NONE',  ( -9.285407649390574392, -287.8515147177142808, -202.3164850531241257 ) ) ;
#1736=CARTESIAN_POINT ( 'NONE',  ( 17.89139397278936272, -287.6724992839841661, -222.3829245675862296 ) ) ;
#1738=CARTESIAN_POINT ( 'NONE',  ( -16.92769768841934308, -296.7698506742665927, -342.9525830315375856 ) ) ;
#1740=CARTESIAN_POINT ( 'NONE',  ( -67.88140272164058331, -290.6492842725307924, -340.6130594856963398 ) ) ;
#1741=CARTESIAN_POINT ( 'NONE',  ( -83.53826820392886532, -277.4427159650949193, -210.7612128747612701 ) ) ;
#1742=CARTESIAN_POINT ( 'NONE',  ( -107.5550754441970440, -278.4808297995886051, -302.0475220878240634 ) ) ;
#1743=CARTESIAN_POINT ( 'NONE',  ( -59.29205138593874835, -279.4422652223107661, -196.5781499539828587 ) ) ;
#1744=CARTESIAN_POINT ( 'NONE',  ( -111.6275770537671264, -274.5438608122422011, -264.8303458579267726 ) ) ;
#1745=CARTESIAN_POINT ( 'NONE',  ( -110.8852626855045571, -282.7408513014555069, -255.6524450881647113 ) ) ;
#1747=CARTESIAN_POINT ( 'NONE',  ( -32.86525229271969550, -278.2487364192615473, -196.2610039735248790 ) ) ;
#1748=CARTESIAN_POINT ( 'NONE',  ( -47.02406441949805327, -281.1749854335209307, -344.7335084835086718 ) ) ;
#1750=CARTESIAN_POINT ( 'NONE',  ( 34.54124994593603049, -274.3598898357928988, -296.1204461415946980 ) ) ;
#1752=CARTESIAN_POINT ( 'NONE',  ( -95.00583646348886191, -298.7141436636807157, -224.4747895665826150 ) ) ;
#1753=CARTESIAN_POINT ( 'NONE',  ( -113.8424131155087764, -283.5491046231293240, -264.2590879456490711 ) ) ;
#1754=CARTESIAN_POINT ( 'NONE',  ( -105.5705267591125249, -273.7087470362338308, -243.8124391693121424 ) ) ;
#1755=CARTESIAN_POINT ( 'NONE',  ( -71.15848572856612009, -275.0397685359516231, -201.8408194792957033 ) ) ;
#1756=CARTESIAN_POINT ( 'NONE',  ( 32.91704035997975808, -275.4823496738562199, -290.3015106855962131 ) ) ;
#1757=CARTESIAN_POINT ( 'NONE',  ( -74.26544743721966313, -297.5432225604704399, -335.6423368310926207 ) ) ;
#1758=CARTESIAN_POINT ( 'NONE',  ( -70.63714881898405906, -289.6457532169164892, -339.8047985140610194 ) ) ;
#1759=CARTESIAN_POINT ( 'NONE',  ( -96.55293578398048737, -277.2721440031359066, -223.4213291589378230 ) ) ;
#1760=CARTESIAN_POINT ( 'NONE',  ( -106.5144451201724678, -289.9497529572378767, -304.3073330078760819 ) ) ;
#1764=CARTESIAN_POINT ( 'NONE',  ( -108.5820832139279304, -289.3876441017661705, -287.3380513535951195 ) ) ;
#1765=CARTESIAN_POINT ( 'NONE',  ( 35.82698505982688886, -291.7642438145344954, -286.8915267809055081 ) ) ;
#1766=ORIENTED_EDGE ( 'NONE', *, *, #4077, .T. ) ;
#1768=CARTESIAN_POINT ( 'NONE',  ( -106.0925958599700465, -289.7307947647781248, -295.0856559489138249 ) ) ;
#1770=CARTESIAN_POINT ( 'NONE',  ( 1.392570185844214992, -287.4976627473723738, -204.0700665931116475 ) ) ;
#1771=CARTESIAN_POINT ( 'NONE',  ( -102.0455923789670294, -293.4805209788416391, -239.2376011013261916 ) ) ;
#1772=CARTESIAN_POINT ( 'NONE',  ( 27.89960822025720688, -293.1427056974741845, -310.9133012240417884 ) ) ;
#1773=CARTESIAN_POINT ( 'NONE',  ( 23.02420457184907931, -283.4994896818116672, -317.3850154914642872 ) ) ;
#1774=CARTESIAN_POINT ( 'NONE',  ( -106.5316306012337861, -284.6965418625353550, -246.9272506044068507 ) ) ;
#1775=CARTESIAN_POINT ( 'NONE',  ( 35.50714259502728964, -276.7400963198646764, -260.6508351919949291 ) ) ;
#1776=CARTESIAN_POINT ( 'NONE',  ( 14.05351214020076256, -290.7980791656141832, -216.2281432195725870 ) ) ;
#1777=CARTESIAN_POINT ( 'NONE',  ( -59.58142725297764031, -272.5526756193522147, -200.3613257485492909 ) ) ;
#1779=CARTESIAN_POINT ( 'NONE',  ( 197.0349383350915105, 285.8449894349855640, -111.9383547020201064 ) ) ;
#1780=CARTESIAN_POINT ( 'NONE',  ( 36.34821029528860237, -293.5004040039983124, -292.8024142208167291 ) ) ;
#1781=CARTESIAN_POINT ( 'NONE',  ( -69.41714365519545993, -287.5468926363182049, -203.1720575300506368 ) ) ;
#1782=CARTESIAN_POINT ( 'NONE',  ( -97.11410897010547671, -298.2783381992039722, -222.3116470947955747 ) ) ;
#1784=CARTESIAN_POINT ( 'NONE',  ( 0.2139193248535528891, -287.2176141071593634, -207.5847406664543939 ) ) ;
#1785=CARTESIAN_POINT ( 'NONE',  ( -110.4462887999276006, -277.3135881266629212, -293.9532670338982712 ) ) ;
#1786=CARTESIAN_POINT ( 'NONE',  ( 36.60385736321685357, -293.9381248450672501, -249.2094290896874895 ) ) ;
#1787=CARTESIAN_POINT ( 'NONE',  ( 6.843122370839409996, -284.7854164591011568, -208.7497002104346677 ) ) ;
#1788=CARTESIAN_POINT ( 'NONE',  ( 39.58590878396767465, -293.9205655783236466, -273.1695478845242064 ) ) ;
#1789=CARTESIAN_POINT ( 'NONE',  ( -38.90228509564093429, -292.3653207151177753, -197.3566519450759245 ) ) ;
#1793=CARTESIAN_POINT ( 'NONE',  ( -111.1989583166938615, -285.8294593436967261, -289.5913245281645914 ) ) ;
#1794=CARTESIAN_POINT ( 'NONE',  ( -2.602324593224659921, -289.9809262143061233, -198.2974183793908196 ) ) ;
#1796=CARTESIAN_POINT ( 'NONE',  ( -100.6750664868626473, -282.9679147868390601, -307.2814481363535606 ) ) ;
#1797=CARTESIAN_POINT ( 'NONE',  ( -112.3801697928137457, -278.4337261398576970, -253.1863585357417321 ) ) ;
#1798=CARTESIAN_POINT ( 'NONE',  ( 33.98635713539291459, -283.8470210494004959, -293.1649254477694058 ) ) ;
#1799=CARTESIAN_POINT ( 'NONE',  ( -68.75627247708085577, -197.2056770039593800, -358.9513570765641362 ) ) ;
#1800=CARTESIAN_POINT ( 'NONE',  ( -102.0100645232851235, -283.6639919249153081, -229.6596568464721884 ) ) ;
#1801=CARTESIAN_POINT ( 'NONE',  ( -33.12099484864842935, -284.1255411062354597, -195.7847949867546333 ) ) ;
#1802=CARTESIAN_POINT ( 'NONE',  ( -73.37858195186689159, -275.4402094594785240, -203.6570937117227516 ) ) ;
#1803=CARTESIAN_POINT ( 'NONE',  ( -103.7771577347053409, -297.4556265425305810, -239.8367178318573849 ) ) ;
#1804=CARTESIAN_POINT ( 'NONE',  ( -9.056457237376076108, -293.3591745649421227, -338.2068753026957211 ) ) ;
#1805=CARTESIAN_POINT ( 'NONE',  ( -100.3771874552530221, -278.6205601094512758, -314.4047341385949039 ) ) ;
#1806=CARTESIAN_POINT ( 'NONE',  ( -5.066084614251986196, -276.6150721985752057, -335.8523681797399263 ) ) ;
#1807=CARTESIAN_POINT ( 'NONE',  ( -29.10309227451535463, -299.0941803680265707, -193.5951300305619327 ) ) ;
#1808=CARTESIAN_POINT ( 'NONE',  ( -41.38196488513791849, -276.0222064098941814, -346.9586636101758472 ) ) ;
#1810=CARTESIAN_POINT ( 'NONE',  ( 1.642048719780067723, -274.5311979272196368, -334.4928091907234489 ) ) ;
#1811=CARTESIAN_POINT ( 'NONE',  ( -94.20088447847305702, -297.2792722567077135, -321.4260710656061519 ) ) ;
#1816=CARTESIAN_POINT ( 'NONE',  ( -51.06232668424904375, -284.3111810020899384, -342.4265939081700481 ) ) ;
#1817=CARTESIAN_POINT ( 'NONE',  ( -58.18695516619104069, -285.0779114967170926, -343.4874171420436824 ) ) ;
#1818=CARTESIAN_POINT ( 'NONE',  ( 26.46039246488074070, -286.4121096519637035, -234.5758016373251280 ) ) ;
#1819=CARTESIAN_POINT ( 'NONE',  ( -109.9151448130932636, -277.1268606013946396, -256.9620305849495026 ) ) ;
#1820=CARTESIAN_POINT ( 'NONE',  ( -108.1571726745488746, -286.1222769201293090, -292.6329461194868031 ) ) ;
#1821=CARTESIAN_POINT ( 'NONE',  ( -94.46582077498722185, -277.6848769671270816, -223.8042431424522931 ) ) ;
#1822=CARTESIAN_POINT ( 'NONE',  ( -69.37412025191891018, -278.5634823524354147, -336.3155171318732073 ) ) ;
#1824=CARTESIAN_POINT ( 'NONE',  ( -89.29032893170928276, -273.7885074658303779, -218.9867235136785553 ) ) ;
#1825=CARTESIAN_POINT ( 'NONE',  ( 30.93834349328282229, -282.8102028399933943, -305.6030598001290173 ) ) ;
#1826=CARTESIAN_POINT ( 'NONE',  ( 4.517479994103495322, -282.9962868592525069, -334.9789950446512989 ) ) ;
#1830=CARTESIAN_POINT ( 'NONE',  ( 25.32221201533798194, -288.8416344733199139, -227.7522788152095927 ) ) ;
#1832=CARTESIAN_POINT ( 'NONE',  ( -94.57125394193877810, -296.3915653539483515, -224.7828348002563814 ) ) ;
#1833=CARTESIAN_POINT ( 'NONE',  ( 23.89908980660779747, -292.2799524007357945, -223.8326897184352049 ) ) ;
#1834=CARTESIAN_POINT ( 'NONE',  ( 34.38961951593933719, -285.8105842117641373, -253.4149402577371006 ) ) ;
#1835=CARTESIAN_POINT ( 'NONE',  ( -82.92535760314615345, -288.2647439289552835, -328.1322620478383669 ) ) ;
#1836=CARTESIAN_POINT ( 'NONE',  ( -11.89864875897552565, -287.5959707400330103, -201.5150458956920829 ) ) ;
#1837=CARTESIAN_POINT ( 'NONE',  ( -110.8389557672072527, -276.3593710714950475, -285.3630322165855659 ) ) ;
#1838=CARTESIAN_POINT ( 'NONE',  ( 19.01866782242020193, -286.6565357626554373, -321.6635789817046316 ) ) ;
#1839=CARTESIAN_POINT ( 'NONE',  ( 24.68852241357335942, -288.9813564656793687, -228.1807187303758440 ) ) ;
#1840=CARTESIAN_POINT ( 'NONE',  ( -43.06863983722212197, -287.1241451343416884, -345.3093040083568894 ) ) ;
#1841=CARTESIAN_POINT ( 'NONE',  ( 16.00545805336161465, -283.2140681170793641, -320.6088823929226237 ) ) ;
#1842=CARTESIAN_POINT ( 'NONE',  ( -89.53178805703595344, -293.3193760021130743, -216.1942795588795718 ) ) ;
#1843=CARTESIAN_POINT ( 'NONE',  ( 82.12427740513938090, -301.4850002582832076, -194.7971909733571465 ) ) ;
#1845=CARTESIAN_POINT ( 'NONE',  ( -111.1924547142390480, -298.2686324635848223, -286.3417390321903326 ) ) ;
#1846=CARTESIAN_POINT ( 'NONE',  ( 23.82313755043268699, -280.1929156344815510, -230.1266894730004253 ) ) ;
#1847=CARTESIAN_POINT ( 'NONE',  ( 32.17914147324426466, -279.9187893134987348, -298.5010047866445575 ) ) ;
#1848=CARTESIAN_POINT ( 'NONE',  ( 38.44531723469279427, -292.9090891060177455, -283.1091178266061661 ) ) ;
#1849=CARTESIAN_POINT ( 'NONE',  ( -93.67062233099235868, -271.4657820610185581, -222.3308699401059698 ) ) ;
#1850=CARTESIAN_POINT ( 'NONE',  ( 34.27671884510021272, -273.8957331200357999, -290.7083564287921718 ) ) ;
#1851=CARTESIAN_POINT ( 'NONE',  ( -94.31428307769847663, -297.2143428639839726, -316.8068356223033106 ) ) ;
#1852=CARTESIAN_POINT ( 'NONE',  ( -96.46848757314708678, -271.7819539807804858, -221.9399898264381648 ) ) ;
#1853=CARTESIAN_POINT ( 'NONE',  ( -109.8394696117295126, -295.0838166859329021, -247.4262068561842227 ) ) ;
#1854=CARTESIAN_POINT ( 'NONE',  ( 17.53195956483178009, -295.6733726494643406, -319.4133392857546028 ) ) ;
#1856=CARTESIAN_POINT ( 'NONE',  ( 21.92953655819888681, -293.7560323184541176, -227.4501664748423764 ) ) ;
#1857=CARTESIAN_POINT ( 'NONE',  ( 82.64890176555634582, -299.5541904835127980, -195.3611179825600175 ) ) ;
#1858=CARTESIAN_POINT ( 'NONE',  ( -72.81592691475427159, -283.6051548763372807, -203.8203578936656868 ) ) ;
#1859=CARTESIAN_POINT ( 'NONE',  ( -95.60433081934026234, -295.9340658417783061, -314.3642732270483293 ) ) ;
#1860=CARTESIAN_POINT ( 'NONE',  ( -105.7841473901820422, -284.0961375919898728, -305.7567879993230804 ) ) ;
#1861=CARTESIAN_POINT ( 'NONE',  ( 35.58859047254066610, -283.2195487465161818, -250.5513702828071132 ) ) ;
#1862=CARTESIAN_POINT ( 'NONE',  ( -35.14458656851743257, -285.7457197627905430, -193.4004832215970282 ) ) ;
#1863=CARTESIAN_POINT ( 'NONE',  ( -107.4187059640009920, -288.8953773174212643, -243.9608039593103967 ) ) ;
#1864=CARTESIAN_POINT ( 'NONE',  ( -54.42813229853332757, -271.3380690714489560, -195.3538533559490702 ) ) ;
#1865=CARTESIAN_POINT ( 'NONE',  ( -35.90716019710459506, -284.7553419901889242, -196.8819673709639062 ) ) ;
#1866=CARTESIAN_POINT ( 'NONE',  ( -70.51784693657312175, -288.3996036156115110, -339.5191348611854210 ) ) ;
#1868=CARTESIAN_POINT ( 'NONE',  ( -109.0718056553745186, -297.9251130639506187, -287.7703970369654485 ) ) ;
#1869=CARTESIAN_POINT ( 'NONE',  ( -113.1350557789254196, -280.1046753220382470, -260.2638623962227484 ) ) ;
#1870=CARTESIAN_POINT ( 'NONE',  ( -36.32253863583939335, -293.0595834506718802, -345.7222541343576836 ) ) ;
#1871=CARTESIAN_POINT ( 'NONE',  ( 4.938849726082819913, -280.3081393567618989, -210.8258965525135409 ) ) ;
#1872=CARTESIAN_POINT ( 'NONE',  ( 23.17299005405337908, -294.3557628267265045, -317.9950054099700765 ) ) ;
#1873=CARTESIAN_POINT ( 'NONE',  ( -112.9154323579523975, -282.6011897958714485, -272.7783060923707694 ) ) ;
#1874=CARTESIAN_POINT ( 'NONE',  ( -112.3774048961945198, -280.5723370782346819, -268.8019203644975050 ) ) ;
#1875=CARTESIAN_POINT ( 'NONE',  ( -28.88065716900909408, -294.0011428959697355, -343.1571866385416456 ) ) ;
#1877=CARTESIAN_POINT ( 'NONE',  ( 72.74377771393429271, -297.4299603653872168, -195.3986477740726571 ) ) ;
#1880=CIRCLE ( 'NONE', #15465, 1.897123461337413275 ) ;
#1881=CARTESIAN_POINT ( 'NONE',  ( -2.401004102695674991, -282.4966363137678513, -204.3845538203418357 ) ) ;
#1882=CARTESIAN_POINT ( 'NONE',  ( -108.3603156578023174, -295.8329766546326596, -287.5703708434563168 ) ) ;
#1884=CARTESIAN_POINT ( 'NONE',  ( 10.59707575819633618, -279.9094976428775681, -330.5268031993606428 ) ) ;
#1885=CARTESIAN_POINT ( 'NONE',  ( -78.74592237100219450, -272.7065600718952396, -205.6320734918893152 ) ) ;
#1887=CARTESIAN_POINT ( 'NONE',  ( 38.85778703060388040, -288.9535576762977485, -277.2121345951974263 ) ) ;
#1888=CARTESIAN_POINT ( 'NONE',  ( -81.72736291092070360, -291.2620429128496085, -212.3410244009469068 ) ) ;
#1890=CARTESIAN_POINT ( 'NONE',  ( -19.38416620746206576, -281.8073654388558111, -198.8364195858591756 ) ) ;
#1891=CARTESIAN_POINT ( 'NONE',  ( -31.29424783336095217, -275.7299018712960219, -196.7965199544862571 ) ) ;
#1893=CARTESIAN_POINT ( 'NONE',  ( -68.67897335434874151, -278.4257154487294201, -203.9901468210984206 ) ) ;
#1894=CARTESIAN_POINT ( 'NONE',  ( 19.84959410240758970, -278.2237576180907013, -318.8807688055062499 ) ) ;
#1896=CARTESIAN_POINT ( 'NONE',  ( 20.03728855721349689, -274.6883701056705718, -218.9344227371128113 ) ) ;
#1897=CARTESIAN_POINT ( 'NONE',  ( -90.86842919715634537, -293.2053341827048598, -218.6290827174546223 ) ) ;
#1898=DIRECTION ( 'NONE',  ( -1.000000000000000000, -0.000000000000000000, -0.000000000000000000 ) ) ;
#1901=CARTESIAN_POINT ( 'NONE',  ( 14.60873643673612676, -290.9132248203426911, -215.1396494589304211 ) ) ;
#1902=CARTESIAN_POINT ( 'NONE',  ( -65.57697277464507124, -297.3391754524017756, -203.0197720991061487 ) ) ;
#1904=CARTESIAN_POINT ( 'NONE',  ( -6.187879255811044032, -293.9742057759335125, -200.6896045566093107 ) ) ;
#1905=CARTESIAN_POINT ( 'NONE',  ( -20.25526795762937127, -276.7662352645559167, -195.3538533559490702 ) ) ;
#1906=CARTESIAN_POINT ( 'NONE',  ( 35.78217053628306843, -289.3476537067894014, -254.4574086725481834 ) ) ;
#1907=CARTESIAN_POINT ( 'NONE',  ( 20.58495107737903496, -274.2066185441614721, -317.7577882374013143 ) ) ;
#1908=CARTESIAN_POINT ( 'NONE',  ( 26.49844309758927707, -276.9546802578913116, -231.9762101116281769 ) ) ;
#1909=CARTESIAN_POINT ( 'NONE',  ( 19.59345793328936480, -290.9639099877106787, -222.4059099524203589 ) ) ;
#1910=CARTESIAN_POINT ( 'NONE',  ( -45.16969867192311483, -281.8145663304621849, -194.9496519062343225 ) ) ;
#1912=CARTESIAN_POINT ( 'NONE',  ( -67.83443920917248704, -282.8118873294255309, -336.7997026443087520 ) ) ;
#1913=CARTESIAN_POINT ( 'NONE',  ( -71.42108493270252723, -278.5713655525021295, -339.0640148827815210 ) ) ;
#1914=CARTESIAN_POINT ( 'NONE',  ( -38.74076183257472650, -281.8642647045426770, -346.9512697412765192 ) ) ;
#1915=CARTESIAN_POINT ( 'NONE',  ( -48.44806128341126339, -278.1313398783293565, -346.3718670637045420 ) ) ;
#1916=CARTESIAN_POINT ( 'NONE',  ( 39.01381927215583545, -277.0821662604436710, -271.1450238814580302 ) ) ;
#1917=CARTESIAN_POINT ( 'NONE',  ( -21.39648532958013050, -294.7662352645559736, -200.3538533559491555 ) ) ;
#1919=CARTESIAN_POINT ( 'NONE',  ( -103.2120358628387038, -298.0758436231525366, -306.2233476429284451 ) ) ;
#1920=CARTESIAN_POINT ( 'NONE',  ( -53.46318296759645250, -290.3435385386808321, -341.8756190553006604 ) ) ;
#1921=CARTESIAN_POINT ( 'NONE',  ( -103.3223180562658854, -276.1072893575904459, -305.2667745100243906 ) ) ;
#1922=CARTESIAN_POINT ( 'NONE',  ( -97.34544202693207637, -291.6813317710332285, -316.9821966407765217 ) ) ;
#1923=CARTESIAN_POINT ( 'NONE',  ( -52.38265163569526095, -291.2031314741498704, -198.7713067025153748 ) ) ;
#1924=CARTESIAN_POINT ( 'NONE',  ( 0.6834181077674537086, -288.0672774831495531, -337.3064253655680318 ) ) ;
#1926=CARTESIAN_POINT ( 'NONE',  ( -92.27400092603585335, -282.2541756316520605, -319.6638362964998805 ) ) ;
#1927=CARTESIAN_POINT ( 'NONE',  ( -111.6040573325567635, -292.4373244364466586, -268.4532604835364396 ) ) ;
#1928=CARTESIAN_POINT ( 'NONE',  ( -99.62730959340170500, -282.4917718055924070, -309.8420990877393706 ) ) ;
#1929=CARTESIAN_POINT ( 'NONE',  ( 24.08557108479768516, -282.3105806660759072, -229.9217102993035837 ) ) ;
#1930=CARTESIAN_POINT ( 'NONE',  ( -96.20289959529432622, -290.8279826483581019, -319.6580630310674564 ) ) ;
#1931=CARTESIAN_POINT ( 'NONE',  ( -100.8684032164926094, -279.5383306389525160, -234.2730806816644531 ) ) ;
#1932=CARTESIAN_POINT ( 'NONE',  ( -42.01433136976206129, -290.7894136091798600, -193.9008326300244391 ) ) ;
#1933=CARTESIAN_POINT ( 'NONE',  ( 0.1959575774732144893, -287.3416398683646094, -203.3007221444231334 ) ) ;
#1934=CARTESIAN_POINT ( 'NONE',  ( 36.32828523687043543, -288.3237080016547793, -292.5938250956721163 ) ) ;
#1935=CARTESIAN_POINT ( 'NONE',  ( -109.6125242434319631, -284.8546033590928914, -260.0689857353383445 ) ) ;
#1938=CARTESIAN_POINT ( 'NONE',  ( 37.10702458874491327, -295.2338532478886464, -256.3007883043370612 ) ) ;
#1939=CARTESIAN_POINT ( 'NONE',  ( 8.596599729177000881, -293.1221787080729086, -331.5409420889323542 ) ) ;
#1940=CARTESIAN_POINT ( 'NONE',  ( -37.82329950544600905, -276.1170400994602119, -343.6073223787289521 ) ) ;
#1941=CARTESIAN_POINT ( 'NONE',  ( -107.6764350356030349, -296.2993689792376131, -239.1435218707934496 ) ) ;
#1942=CARTESIAN_POINT ( 'NONE',  ( 31.22360272392403147, -292.3914795338272370, -297.5100297038638928 ) ) ;
#1943=CARTESIAN_POINT ( 'NONE',  ( -68.45332359307698766, -295.8775789098493192, -203.1904272105183225 ) ) ;
#1945=CARTESIAN_POINT ( 'NONE',  ( -3.466565670280920664, -293.7149322609615183, -205.2488628282713705 ) ) ;
#1946=CARTESIAN_POINT ( 'NONE',  ( 30.13490306836979471, -294.2471641990571811, -241.5758669598086215 ) ) ;
#1949=CARTESIAN_POINT ( 'NONE',  ( -9.101046344283929557, -292.6837187558634810, -340.0760895588767880 ) ) ;
#1950=CARTESIAN_POINT ( 'NONE',  ( -82.28888259837283670, -299.4394134775402563, -210.2575296171674495 ) ) ;
#1951=CARTESIAN_POINT ( 'NONE',  ( 33.31208926155937178, -288.7494412400940291, -289.8224719517164090 ) ) ;
#1956=CARTESIAN_POINT ( 'NONE',  ( 15.81326990028412283, -278.2842661999981146, -323.8470756747084351 ) ) ;
#1957=CARTESIAN_POINT ( 'NONE',  ( -67.15474507633625478, -278.3541955935785381, -199.9020474208194855 ) ) ;
#1959=CARTESIAN_POINT ( 'NONE',  ( -106.7476530637889169, -272.3257423396635772, -237.2533170384528773 ) ) ;
#1960=CARTESIAN_POINT ( 'NONE',  ( -5.437532595103494515, -280.7090473537692219, -337.6316490276136619 ) ) ;
#1961=CARTESIAN_POINT ( 'NONE',  ( -72.12328436148176536, -277.9998443741489496, -202.5477870108646528 ) ) ;
#1963=CARTESIAN_POINT ( 'NONE',  ( -109.6302219920987540, -295.0624182200518817, -283.6828267874411154 ) ) ;
#1964=CARTESIAN_POINT ( 'NONE',  ( -87.02632044705406145, -275.3610118057939076, -214.1103711793309969 ) ) ;
#1965=CARTESIAN_POINT ( 'NONE',  ( -31.33959885877072438, -274.7813397628189591, -197.4933380385196529 ) ) ;
#1967=CARTESIAN_POINT ( 'NONE',  ( -101.7956337022391722, -289.0941016233005598, -231.2208794897481425 ) ) ;
#1968=CARTESIAN_POINT ( 'NONE',  ( -75.66368098456607072, -289.5489432952361994, -337.1475371352232173 ) ) ;
#1969=CARTESIAN_POINT ( 'NONE',  ( -46.67911778174227777, -275.9340286220564167, -195.7766621180727498 ) ) ;
#1970=CARTESIAN_POINT ( 'NONE',  ( -96.72882652426994810, -295.1771302697427473, -224.8078669088284016 ) ) ;
#1971=CARTESIAN_POINT ( 'NONE',  ( -4.242673219856334832, -281.8240457468197633, -339.7197407501331554 ) ) ;
#1973=CARTESIAN_POINT ( 'NONE',  ( 22.03161527036013112, -280.1801386287440323, -316.2054480051863266 ) ) ;
#1976=CARTESIAN_POINT ( 'NONE',  ( -107.7720124723185933, -289.6194163490811775, -249.6597668280071503 ) ) ;
#1977=CARTESIAN_POINT ( 'NONE',  ( -35.88588397217707637, -284.2101882754647022, -196.1401904582852751 ) ) ;
#1980=CARTESIAN_POINT ( 'NONE',  ( 37.70920793677652938, -291.5575744195288621, -270.7962710752898943 ) ) ;
#1981=CARTESIAN_POINT ( 'NONE',  ( -36.43613440273270498, -278.6407826863052151, -344.1681683069380142 ) ) ;
#1982=CARTESIAN_POINT ( 'NONE',  ( -0.5525842283535833399, -283.7795395071905205, -337.5665288592011279 ) ) ;
#1983=CARTESIAN_POINT ( 'NONE',  ( 22.50752180093631338, -273.0045209359668661, -224.2164673674942890 ) ) ;
#1984=CARTESIAN_POINT ( 'NONE',  ( -39.97391833633340497, -286.0181600753365387, -197.4085893951001367 ) ) ;
#1985=CARTESIAN_POINT ( 'NONE',  ( 17.88938769955537111, -277.6664278175513800, -319.0103906305160422 ) ) ;
#1986=CARTESIAN_POINT ( 'NONE',  ( -43.20987102546752112, -277.9309823070757375, -343.2868767880636938 ) ) ;
#1987=CARTESIAN_POINT ( 'NONE',  ( -80.39215963328472014, -285.6351848317096369, -331.8381158696838042 ) ) ;
#1989=DIRECTION ( 'NONE',  ( 0.01273136352371030157, 0.9999189529070979798, 0.000000000000000000 ) ) ;
#1990=CARTESIAN_POINT ( 'NONE',  ( -86.39694989274904913, -295.5451879507772901, -329.7124656927044839 ) ) ;
#1991=CARTESIAN_POINT ( 'NONE',  ( -3.879320491256792902, -288.4757104310828595, -203.6369397903436038 ) ) ;
#1993=CARTESIAN_POINT ( 'NONE',  ( -88.52914483777347243, -287.1952119285918457, -334.4957818155094174 ) ) ;
#1994=CARTESIAN_POINT ( 'NONE',  ( -111.7825392023984250, -277.7047219313773212, -251.8667266803492168 ) ) ;
#1995=CARTESIAN_POINT ( 'NONE',  ( -101.0042560621475900, -289.5093916096729458, -228.3914229997147629 ) ) ;
#1996=CARTESIAN_POINT ( 'NONE',  ( -81.91315779100871453, -286.9522013627462229, -211.6747233722719557 ) ) ;
#1997=CARTESIAN_POINT ( 'NONE',  ( -110.6283986156055335, -280.4515435532562719, -259.6590341996831057 ) ) ;
#1998=CARTESIAN_POINT ( 'NONE',  ( 17.91276743108515745, -288.2493991783006209, -217.5065192596706538 ) ) ;
#1999=CARTESIAN_POINT ( 'NONE',  ( -3.913476057354651427, -284.6113574538759394, -337.4994415272765309 ) ) ;
#2000=CARTESIAN_POINT ( 'NONE',  ( -11.86418208911024053, -276.8962747227436125, -343.0799387615849128 ) ) ;
#2001=CARTESIAN_POINT ( 'NONE',  ( -107.1166455203094472, -270.9062053245839934, -243.1723182243472365 ) ) ;
#2002=CARTESIAN_POINT ( 'NONE',  ( -42.42793438594448219, -279.8229892678264719, -193.5292871727605757 ) ) ;
#2004=CARTESIAN_POINT ( 'NONE',  ( -44.73598588289178224, -299.8781409322182867, -196.2378934212745207 ) ) ;
#2006=CARTESIAN_POINT ( 'NONE',  ( -4.829096099716510437, -282.9805209788416391, -202.7746430608542312 ) ) ;
#2007=CARTESIAN_POINT ( 'NONE',  ( 19.29575570832072273, -273.0951662187703732, -219.6263609375178589 ) ) ;
#2008=DIRECTION ( 'NONE',  ( -1.000000000000000000, -0.000000000000000000, -0.000000000000000000 ) ) ;
#2010=CARTESIAN_POINT ( 'NONE',  ( -61.81634175569918455, -276.8865265792036894, -339.2551582312770506 ) ) ;
#2012=CARTESIAN_POINT ( 'NONE',  ( -41.18826645213862037, -275.2099551193472848, -193.8028367402565095 ) ) ;
#2013=CARTESIAN_POINT ( 'NONE',  ( -4.276076615609534670, -281.6856487468970727, -339.6538752760456532 ) ) ;
#2014=CARTESIAN_POINT ( 'NONE',  ( -42.71541642840033148, -290.8808796353594630, -344.2304245617198717 ) ) ;
#2015=CARTESIAN_POINT ( 'NONE',  ( -95.05948908248903706, -298.7532897346009690, -220.3686610771193841 ) ) ;
#2016=CARTESIAN_POINT ( 'NONE',  ( -100.4323919280489008, -298.3340155440513968, -226.8918481742781523 ) ) ;
#2017=CARTESIAN_POINT ( 'NONE',  ( 0.8226664419661585681, -294.5626779565457127, -205.9910197163725343 ) ) ;
#2018=CARTESIAN_POINT ( 'NONE',  ( 27.12578989863462553, -280.0623675370210890, -308.4630762548672465 ) ) ;
#2020=CARTESIAN_POINT ( 'NONE',  ( 20.78542030481310121, -282.8279840764689084, -223.8578700069980414 ) ) ;
#2021=CARTESIAN_POINT ( 'NONE',  ( -67.70395980963517957, -271.6718903748085836, -202.1563572596103029 ) ) ;
#2022=CARTESIAN_POINT ( 'NONE',  ( -81.08546537373352692, -285.2352171238882192, -332.8185952326336974 ) ) ;
#2024=CARTESIAN_POINT ( 'NONE',  ( -71.32822682572701467, -288.4322730365837515, -335.3302249025298920 ) ) ;
#2025=CARTESIAN_POINT ( 'NONE',  ( 201.1547583153258358, 288.4971606646042233, -97.45162841053168279 ) ) ;
#2026=ORIENTED_EDGE ( 'NONE', *, *, #60434, .F. ) ;
#2027=CARTESIAN_POINT ( 'NONE',  ( -4.602114273523942423, -287.2039942887722077, -339.4169636361654057 ) ) ;
#2028=CARTESIAN_POINT ( 'NONE',  ( 12.16702034026408263, -288.0074480611583567, -324.1045288833065570 ) ) ;
#2029=ORIENTED_EDGE ( 'NONE', *, *, #54431, .F. ) ;
#2030=CARTESIAN_POINT ( 'NONE',  ( -107.9371932011896575, -285.2473543258305995, -300.4597063634721508 ) ) ;
#2032=CARTESIAN_POINT ( 'NONE',  ( 25.29178249154562153, -275.3680629837697325, -232.7247502308229912 ) ) ;
#2033=CARTESIAN_POINT ( 'NONE',  ( -42.02130980168755059, -290.9147976919833809, -193.8131345778098193 ) ) ;
#2034=CARTESIAN_POINT ( 'NONE',  ( 6.873188760179909096, -283.1195543310718108, -333.3417071995940546 ) ) ;
#2035=CARTESIAN_POINT ( 'NONE',  ( 37.74681026919502358, -283.2445694927249065, -284.0140511247211634 ) ) ;
#2036=CARTESIAN_POINT ( 'NONE',  ( -90.42048600183871088, -284.1120019392710674, -326.1871110726198140 ) ) ;
#2037=CARTESIAN_POINT ( 'NONE',  ( -57.11321054484388782, -279.7898631630807245, -200.0895919151701605 ) ) ;
#2038=CARTESIAN_POINT ( 'NONE',  ( 10.64812456238590777, -272.1952119285918457, -210.2361428286349110 ) ) ;
#2039=CARTESIAN_POINT ( 'NONE',  ( -95.22016405621698709, -240.3877380467951639, -341.9231918056108270 ) ) ;
#2041=CARTESIAN_POINT ( 'NONE',  ( 37.20209665873868943, -277.4604354044789147, -263.2211078531785802 ) ) ;
#2042=CARTESIAN_POINT ( 'NONE',  ( 138.0606683641728409, 180.7651495054645920, -241.0585848927976258 ) ) ;
#2044=CARTESIAN_POINT ( 'NONE',  ( -94.52587752461543857, -296.5429601974807383, -224.8214372187032382 ) ) ;
#2045=CARTESIAN_POINT ( 'NONE',  ( 21.26764366597424072, -292.3870628483946348, -220.4965133666736676 ) ) ;
#2046=CARTESIAN_POINT ( 'NONE',  ( 180.0836269057962795, 251.0244910124412172, -164.3671539780329454 ) ) ;
#2047=CARTESIAN_POINT ( 'NONE',  ( -93.21936848272368081, -295.8435837508641271, -218.1658974459102183 ) ) ;
#2048=CARTESIAN_POINT ( 'NONE',  ( -110.5859630443777775, -288.8340604813959089, -279.4009390329691200 ) ) ;
#2049=CARTESIAN_POINT ( 'NONE',  ( -96.57585051210328686, -297.7941808949692017, -315.1277865623907815 ) ) ;
#2050=CARTESIAN_POINT ( 'NONE',  ( 13.46848417807374254, -288.0963321584071650, -217.1913126699191992 ) ) ;
#2052=CARTESIAN_POINT ( 'NONE',  ( 17.40218351614037573, -295.2351209530521601, -324.2505576784660093 ) ) ;
#2053=CARTESIAN_POINT ( 'NONE',  ( -78.40604531219229045, -284.1139214789589573, -330.7904816738076192 ) ) ;
#2054=CARTESIAN_POINT ( 'NONE',  ( -114.0325882487032914, -271.4726545306050980, -270.3474016006499596 ) ) ;
#2056=CARTESIAN_POINT ( 'NONE',  ( 11.00922700175544833, -293.5044262244004472, -210.5737734599591988 ) ) ;
#2057=CARTESIAN_POINT ( 'NONE',  ( 37.02148816262170072, -293.7965949533668777, -250.5709245253850384 ) ) ;
#2058=CARTESIAN_POINT ( 'NONE',  ( -49.69081312820068774, -292.0570746453730635, -198.3618984261759408 ) ) ;
#2061=CARTESIAN_POINT ( 'NONE',  ( -26.45528139451065286, -300.0474666281319855, -194.5929036537726518 ) ) ;
#2062=CARTESIAN_POINT ( 'NONE',  ( -15.87385002818944280, -273.1186214841131346, -196.7728019898977152 ) ) ;
#2064=CARTESIAN_POINT ( 'NONE',  ( -54.12393806463698809, -276.7696001028011210, -345.5015556906572556 ) ) ;
#2065=CARTESIAN_POINT ( 'NONE',  ( -93.50954456418412519, -271.6257690309754480, -222.4708157400283142 ) ) ;
#2066=CARTESIAN_POINT ( 'NONE',  ( -109.3648041150566570, -280.1785363210345281, -288.4006138067650795 ) ) ;
#2067=CARTESIAN_POINT ( 'NONE',  ( -73.46341564798592572, -275.6762773280892702, -335.2300986960959790 ) ) ;
#2068=CARTESIAN_POINT ( 'NONE',  ( -101.5694060139669546, -298.2401026749955122, -234.8374315116672335 ) ) ;
#2069=CARTESIAN_POINT ( 'NONE',  ( -110.5774403763021212, -273.5291849198071645, -267.6404355218357409 ) ) ;
#2070=CARTESIAN_POINT ( 'NONE',  ( -33.40664285205567552, -299.7007609888386810, -194.1600618764771582 ) ) ;
#2071=CARTESIAN_POINT ( 'NONE',  ( 8.529493450450990721, -272.6970729445243933, -210.5761667032649882 ) ) ;
#2072=CARTESIAN_POINT ( 'NONE',  ( 33.87661159185390858, -294.4214209168420666, -286.9040071116637591 ) ) ;
#2073=CARTESIAN_POINT ( 'NONE',  ( -68.03050189274372883, -290.2158688182970536, -203.4625054185326576 ) ) ;
#2074=DIRECTION ( 'NONE',  ( -1.000000000000000000, -0.000000000000000000, -0.000000000000000000 ) ) ;
#2075=CARTESIAN_POINT ( 'NONE',  ( -48.47887736332177866, -277.6825073734515286, -346.5430856636735939 ) ) ;
#2077=CARTESIAN_POINT ( 'NONE',  ( -24.59852022289694062, -274.3858610515175656, -198.4303855360653301 ) ) ;
#2078=CARTESIAN_POINT ( 'NONE',  ( -112.9971824448755200, -283.3846358296967765, -258.6304402422449584 ) ) ;
#2079=CARTESIAN_POINT ( 'NONE',  ( -98.50159136657043746, -297.9583063324445789, -314.1465297772388112 ) ) ;
#2082=CARTESIAN_POINT ( 'NONE',  ( 11.24892245177460737, -285.9427870572646384, -215.5979501576665598 ) ) ;
#2083=CARTESIAN_POINT ( 'NONE',  ( -34.57263458211485130, -281.0172621161066786, -345.4767668524411874 ) ) ;
#2084=CARTESIAN_POINT ( 'NONE',  ( -36.47651045864730435, -275.2810569442526116, -344.3820383394859164 ) ) ;
#2085=CARTESIAN_POINT ( 'NONE',  ( -35.11786842070824832, -275.5984073651620747, -343.9167397327077538 ) ) ;
#2086=CARTESIAN_POINT ( 'NONE',  ( 30.10818696972672370, -283.9858643997600893, -303.2733891445327004 ) ) ;
#2087=CARTESIAN_POINT ( 'NONE',  ( 35.41208883775818350, -276.6300157962704134, -260.6648972799100648 ) ) ;
#2089=CARTESIAN_POINT ( 'NONE',  ( -106.1123779067414006, -271.3771798491576988, -237.5429173728900878 ) ) ;
#2091=CARTESIAN_POINT ( 'NONE',  ( -9.562898643533312537, -282.4144454992721194, -200.5158130911784440 ) ) ;
#2093=CARTESIAN_POINT ( 'NONE',  ( 19.19276175889717351, -288.7795142148936520, -220.1523971396397314 ) ) ;
#2095=CARTESIAN_POINT ( 'NONE',  ( -107.6956553187080630, -288.8909507053044763, -244.2265189771908354 ) ) ;
#2097=CARTESIAN_POINT ( 'NONE',  ( -90.32191148886263932, -296.0768748765642044, -219.4924588635598468 ) ) ;
#2098=CARTESIAN_POINT ( 'NONE',  ( -102.1913712050967149, -289.1788048894101735, -234.1254742418522596 ) ) ;
#2099=CARTESIAN_POINT ( 'NONE',  ( -107.5887910744927609, -275.4946769126667618, -270.3985833712262092 ) ) ;
#2100=CARTESIAN_POINT ( 'NONE',  ( 54.76408350478209996, -297.2049266773145177, -195.3925142569238744 ) ) ;
#2101=CARTESIAN_POINT ( 'NONE',  ( 19.09826794285438822, -286.7365292651955997, -321.7346180336016346 ) ) ;
#2102=CARTESIAN_POINT ( 'NONE',  ( -21.95339105724425011, -281.0974418033774782, -344.7733075435555747 ) ) ;
#2103=CARTESIAN_POINT ( 'NONE',  ( -92.55649793336425546, -291.2325886586795036, -222.6083578181284395 ) ) ;
#2105=CIRCLE ( 'NONE', #32385, 1.897123461337413275 ) ;
#2106=CARTESIAN_POINT ( 'NONE',  ( 34.63776245489370353, -282.7763513045014179, -254.9932462029766498 ) ) ;
#2107=CARTESIAN_POINT ( 'NONE',  ( -13.46703237403166042, -283.5370432515453558, -339.5712027365387371 ) ) ;
#2108=CARTESIAN_POINT ( 'NONE',  ( -64.82316766814668085, -291.3890356585741870, -340.5815942037149853 ) ) ;
#2109=CARTESIAN_POINT ( 'NONE',  ( -110.0832714527496279, -273.2030633494566700, -245.1736589463104679 ) ) ;
#2111=CARTESIAN_POINT ( 'NONE',  ( -6.241949309262166068, -286.7265899512405554, -339.2241683085647423 ) ) ;
#2112=CARTESIAN_POINT ( 'NONE',  ( 37.63491125693305150, -275.3321891305067197, -252.7678633170977207 ) ) ;
#2113=CARTESIAN_POINT ( 'NONE',  ( -84.89585910391330970, -293.3723453931884251, -212.8246185782433315 ) ) ;
#2115=CARTESIAN_POINT ( 'NONE',  ( -54.42813229853333468, -279.7662352645560304, -345.3683826091709648 ) ) ;
#2116=CARTESIAN_POINT ( 'NONE',  ( -51.00496992666680995, -275.2262152499130821, -344.2755514994900068 ) ) ;
#2118=CARTESIAN_POINT ( 'NONE',  ( -67.83836636071875148, -296.0585325629652971, -200.4737381892856831 ) ) ;
#2119=CARTESIAN_POINT ( 'NONE',  ( -99.36258011767341713, -272.4340756826957204, -231.6661168403955742 ) ) ;
#2120=CARTESIAN_POINT ( 'NONE',  ( -70.55032696535013770, -293.1261357774674252, -204.5743802770932689 ) ) ;
#2122=CARTESIAN_POINT ( 'NONE',  ( -105.9352276611975725, -291.8363160362087001, -244.5590881221161226 ) ) ;
#2123=CARTESIAN_POINT ( 'NONE',  ( -92.40412902279267371, -285.6139025892744598, -319.8382743476557266 ) ) ;
#2124=CARTESIAN_POINT ( 'NONE',  ( 37.21304882180386642, -295.1891219558214630, -287.1592840552299890 ) ) ;
#2125=CARTESIAN_POINT ( 'NONE',  ( 30.45410925536853242, -294.4056411055672697, -234.7925460162518050 ) ) ;
#2126=CARTESIAN_POINT ( 'NONE',  ( 17.97104195241555757, -294.0641211834099522, -318.0194522114629194 ) ) ;
#2127=CARTESIAN_POINT ( 'NONE',  ( 37.63039947879230596, -289.5968253745170955, -273.8275428787123928 ) ) ;
#2128=CARTESIAN_POINT ( 'NONE',  ( 9.210491383358622386, -282.5990530749176628, -331.6953944514881414 ) ) ;
#2129=CARTESIAN_POINT ( 'NONE',  ( -15.30887110482980340, -296.4057675595481101, -194.8082513318286146 ) ) ;
#2130=CARTESIAN_POINT ( 'NONE',  ( -80.93645673547408137, -285.3117699972636956, -206.8263170742234536 ) ) ;
#2131=CARTESIAN_POINT ( 'NONE',  ( 6.380162456785919645, -278.4353498808865766, -330.9249243190263883 ) ) ;
#2132=CARTESIAN_POINT ( 'NONE',  ( -110.7057658001759819, -283.3759472869606384, -268.1601246309364797 ) ) ;
#2133=CARTESIAN_POINT ( 'NONE',  ( 37.35323648695389664, -285.6387572774202681, -277.1188610237232979 ) ) ;
#2134=CARTESIAN_POINT ( 'NONE',  ( -92.16335732991835528, -277.4191286299256376, -217.9899962859443860 ) ) ;
#2136=CARTESIAN_POINT ( 'NONE',  ( -85.76224650306876640, -284.8681506636110612, -215.5811734984633290 ) ) ;
#2137=CARTESIAN_POINT ( 'NONE',  ( -38.18102986284067413, -281.2469223001485830, -193.7627874137964454 ) ) ;
#2138=CARTESIAN_POINT ( 'NONE',  ( 37.27287069503110217, -286.8378896028766007, -288.4578431553505311 ) ) ;
#2139=CARTESIAN_POINT ( 'NONE',  ( -5.079819362040934649, -296.3816686781034377, -336.9870216331694905 ) ) ;
#2140=CARTESIAN_POINT ( 'NONE',  ( -62.12632313572955667, -278.9691406889381255, -342.4734999533521886 ) ) ;
#2141=CARTESIAN_POINT ( 'NONE',  ( -97.53050330547524993, -279.2318537549370490, -317.5904123559145091 ) ) ;
#2142=CARTESIAN_POINT ( 'NONE',  ( -101.8579128402041647, -277.9202096510903743, -304.5174980859699190 ) ) ;
#2143=CARTESIAN_POINT ( 'NONE',  ( -95.04310408981875469, -299.2114048706596350, -222.6906102932771887 ) ) ;
#2144=CARTESIAN_POINT ( 'NONE',  ( -19.35104256547869639, -284.2839792348823380, -197.7225286248480813 ) ) ;
#2145=CARTESIAN_POINT ( 'NONE',  ( -112.3877150568496290, -292.3192350521095477, -257.1499083572876430 ) ) ;
#2146=CARTESIAN_POINT ( 'NONE',  ( 14.52530201901463691, -293.2218347199890331, -322.2402020043435300 ) ) ;
#2148=CARTESIAN_POINT ( 'NONE',  ( 33.13599404509604796, -293.4717298116592588, -289.5131541331921881 ) ) ;
#2149=CARTESIAN_POINT ( 'NONE',  ( -112.8699938290462654, -291.7988621492231687, -257.0581348260722052 ) ) ;
#2150=CARTESIAN_POINT ( 'NONE',  ( -74.56482774962780979, -280.1945662622522946, -207.3876600772935888 ) ) ;
#2151=CARTESIAN_POINT ( 'NONE',  ( -97.62083320307297640, -272.2486007453424577, -222.8295881325881851 ) ) ;
#2152=CARTESIAN_POINT ( 'NONE',  ( 36.68853772482916042, -288.4651707061570391, -291.2141542374308187 ) ) ;
#2153=CARTESIAN_POINT ( 'NONE',  ( 25.83678602795502854, -288.4678089045153797, -314.4324517823617384 ) ) ;
#2154=CARTESIAN_POINT ( 'NONE',  ( 0.1758841609052546329, -286.8995333785741764, -207.6561946568479868 ) ) ;
#2157=CARTESIAN_POINT ( 'NONE',  ( 201.3567858607021606, 295.1816420246623238, -54.00000000001949019 ) ) ;
#2158=CARTESIAN_POINT ( 'NONE',  ( 198.2830375120520046, 286.1211273803923518, -96.28769358250616506 ) ) ;
#2159=CARTESIAN_POINT ( 'NONE',  ( -18.98628338888636335, -276.0069143675299301, -341.1825864986541319 ) ) ;
#2160=CARTESIAN_POINT ( 'NONE',  ( -105.7980234881359252, -277.8229843096455056, -243.9900548994116321 ) ) ;
#2161=CARTESIAN_POINT ( 'NONE',  ( -34.04393657811251472, -297.6000597370594392, -193.4229229018398541 ) ) ;
#2162=CARTESIAN_POINT ( 'NONE',  ( -29.26882874936469037, -125.6146630139821951, -361.3924731419004388 ) ) ;
#2163=CARTESIAN_POINT ( 'NONE',  ( -88.89226258380361401, -276.4434881388031613, -326.8928593510478890 ) ) ;
#2165=CARTESIAN_POINT ( 'NONE',  ( -50.27273100689873075, -296.9750370634604337, -345.2926686585216203 ) ) ;
#2166=CARTESIAN_POINT ( 'NONE',  ( -82.57946348516480839, -290.1820548303577993, -327.7330031520684770 ) ) ;
#2167=CARTESIAN_POINT ( 'NONE',  ( -36.55297263512778727, -298.8646194353156602, -193.5224886275879328 ) ) ;
#2168=CARTESIAN_POINT ( 'NONE',  ( -68.80994990612290962, -274.3006431686073370, -200.1822055469266672 ) ) ;
#2169=CARTESIAN_POINT ( 'NONE',  ( -108.2985123843628088, -296.4918970600967327, -287.5640672187727205 ) ) ;
#2172=CONICAL_SURFACE ( 'NONE', #71746, 5.751884811727114410, 0.09862129276975223346 ) ;
#2174=CARTESIAN_POINT ( 'NONE',  ( -107.3135515301804332, -280.1032050792717314, -298.8787302077540744 ) ) ;
#2176=CARTESIAN_POINT ( 'NONE',  ( 28.24925827808030121, -281.5868286147847357, -310.6783973071230207 ) ) ;
#2177=CARTESIAN_POINT ( 'NONE',  ( -97.12986316287404520, -279.0416937208063928, -312.8046259114348686 ) ) ;
#2178=CARTESIAN_POINT ( 'NONE',  ( -113.0672085133617202, -280.2248409079646194, -277.2616554735079717 ) ) ;
#2179=CARTESIAN_POINT ( 'NONE',  ( -37.12983572553468292, -296.6295895495666741, -196.7690653795428091 ) ) ;
#2182=CARTESIAN_POINT ( 'NONE',  ( -1.967936964375852638, -280.7013088756389152, -206.5042711753958145 ) ) ;
#2183=CARTESIAN_POINT ( 'NONE',  ( 37.08489092440437673, -276.5945191054177030, -289.4619390470704161 ) ) ;
#2185=CARTESIAN_POINT ( 'NONE',  ( 29.45714011259948961, -277.1013848038942342, -236.2595698035918872 ) ) ;
#2186=CARTESIAN_POINT ( 'NONE',  ( 35.92328741275411375, -274.4017415834833287, -292.1062735238747905 ) ) ;
#2189=CARTESIAN_POINT ( 'NONE',  ( -90.87037250449097314, -290.4650436712174724, -220.4699305656451713 ) ) ;
#2191=CARTESIAN_POINT ( 'NONE',  ( 7.491243797183925857, -285.9942245840188662, -207.8189745828121602 ) ) ;
#2192=CARTESIAN_POINT ( 'NONE',  ( -83.44318099377669284, -281.9335766161375432, -328.3287769936021618 ) ) ;
#2193=CARTESIAN_POINT ( 'NONE',  ( -45.72447033844620279, -281.7350656210365401, -343.5227434028674907 ) ) ;
#2194=CARTESIAN_POINT ( 'NONE',  ( 0.9295821358342835072, -284.6464615516525214, -206.4525739628948600 ) ) ;
#2195=CARTESIAN_POINT ( 'NONE',  ( 1.454519360038549980, -290.5343190514456069, -334.6069610176664355 ) ) ;
#2196=CARTESIAN_POINT ( 'NONE',  ( 29.32696467460198875, -282.3438574566447983, -239.5405191740171915 ) ) ;
#2197=CARTESIAN_POINT ( 'NONE',  ( -71.48679578107388011, -195.9896643738506157, -360.3036384909707976 ) ) ;
#2198=CARTESIAN_POINT ( 'NONE',  ( -33.12361566198947571, -281.3997657408445434, -346.4572828301221534 ) ) ;
#2199=CARTESIAN_POINT ( 'NONE',  ( 34.46253570979931879, -295.8334690828931457, -292.1971763898333734 ) ) ;
#2200=CARTESIAN_POINT ( 'NONE',  ( -73.26651385536025884, -277.8223967714851597, -203.3883061970796575 ) ) ;
#2201=CARTESIAN_POINT ( 'NONE',  ( -80.87344174830758448, -278.3124224331256755, -329.0882849443885334 ) ) ;
#2202=CARTESIAN_POINT ( 'NONE',  ( -109.9569423336974978, -286.8036344208911146, -250.7473301568039403 ) ) ;
#2204=CARTESIAN_POINT ( 'NONE',  ( -35.02944484669908576, -294.0010962748318661, -194.8235972500390005 ) ) ;
#2205=CARTESIAN_POINT ( 'NONE',  ( 22.41543008159820971, -274.1719576823524562, -315.6831439879010759 ) ) ;
#2206=CARTESIAN_POINT ( 'NONE',  ( -87.28725171546295769, -288.9247472652098736, -328.8227987163301691 ) ) ;
#2207=CARTESIAN_POINT ( 'NONE',  ( 13.46854512744152110, -291.1777817917465541, -216.8376708685118217 ) ) ;
#2209=CARTESIAN_POINT ( 'NONE',  ( -96.49986287289850395, -276.6296810931860364, -313.9890440177367736 ) ) ;
#2210=CARTESIAN_POINT ( 'NONE',  ( -110.4889849235264876, -294.8559942294779148, -257.6985665523233706 ) ) ;
#2211=CARTESIAN_POINT ( 'NONE',  ( -103.2805671625126962, -291.4304952868459395, -302.8158447689691570 ) ) ;
#2214=CARTESIAN_POINT ( 'NONE',  ( 18.91768952103209855, -291.3243543124797270, -218.8093107466258971 ) ) ;
#2215=CARTESIAN_POINT ( 'NONE',  ( 36.25134222208720303, -289.2327586950282239, -276.5281224241958284 ) ) ;
#2216=CARTESIAN_POINT ( 'NONE',  ( -111.9259605917659002, -288.9770328163453996, -255.7620185274782614 ) ) ;
#2217=CARTESIAN_POINT ( 'NONE',  ( 35.71132314271395103, -289.0934693570068248, -279.2285137563272883 ) ) ;
#2218=FACE_OUTER_BOUND ( 'NONE', #21146, .T. ) ;
#2219=CARTESIAN_POINT ( 'NONE',  ( 1.405749720908947120, -289.3226808537093007, -332.4194522901951245 ) ) ;
#2220=CARTESIAN_POINT ( 'NONE',  ( -73.78824644324126325, -297.5130670652411027, -336.3745011791797879 ) ) ;
#2222=CARTESIAN_POINT ( 'NONE',  ( -62.61807503945496478, -290.5788577575258955, -342.7298173787915516 ) ) ;
#2223=CARTESIAN_POINT ( 'NONE',  ( -67.98017750926324254, -277.6720681022069925, -201.5016318467622796 ) ) ;
#2224=CARTESIAN_POINT ( 'NONE',  ( -77.80017677024424927, -277.9127130900238285, -335.9124174681257955 ) ) ;
#2225=CARTESIAN_POINT ( 'NONE',  ( -1.141626563160716090, -280.1859037399913746, -202.4251263030592725 ) ) ;
#2226=CARTESIAN_POINT ( 'NONE',  ( -109.3390285280996892, -274.7195291724283379, -251.2502868355318526 ) ) ;
#2227=CARTESIAN_POINT ( 'NONE',  ( -35.86934699209479049, -284.0704663254091997, -195.3755671829415235 ) ) ;
#2230=CARTESIAN_POINT ( 'NONE',  ( 5.657576158118884813, -278.7812504572832495, -209.8472541431163734 ) ) ;
#2231=CARTESIAN_POINT ( 'NONE',  ( -64.55098927550875487, -281.4071551661360786, -340.2652635527532539 ) ) ;
#2233=CARTESIAN_POINT ( 'NONE',  ( -68.74786636221647029, -275.9373961078078423, -339.9193412242318573 ) ) ;
#2234=CARTESIAN_POINT ( 'NONE',  ( -55.95995789428866374, -296.8162748563663058, -341.7166470610565625 ) ) ;
#2235=CARTESIAN_POINT ( 'NONE',  ( 11.28594217932069554, -281.3170560725138216, -329.7328204633518567 ) ) ;
#2236=CARTESIAN_POINT ( 'NONE',  ( -69.37122856281865779, -298.5612167196425162, -204.5012838102906585 ) ) ;
#2237=CARTESIAN_POINT ( 'NONE',  ( -85.45141967122081894, -274.8269922462721411, -210.9973143917986818 ) ) ;
#2238=CARTESIAN_POINT ( 'NONE',  ( -91.13524100074610601, -272.9275398589860515, -220.9630344600264777 ) ) ;
#2239=CARTESIAN_POINT ( 'NONE',  ( 37.64258315267473165, -295.5932523154244222, -273.5492605342137722 ) ) ;
#2240=CARTESIAN_POINT ( 'NONE',  ( 36.69063261085982219, -287.4512972533717630, -249.0007533794227186 ) ) ;
#2241=CARTESIAN_POINT ( 'NONE',  ( -83.66447488269824362, -277.5024444815465472, -210.5997397295432165 ) ) ;
#2243=CARTESIAN_POINT ( 'NONE',  ( -111.9225647292233674, -290.1452350983350357, -289.5631431920322711 ) ) ;
#2244=CARTESIAN_POINT ( 'NONE',  ( -84.84673796580017324, -288.7846177701384818, -326.1656610729313570 ) ) ;
#2245=CARTESIAN_POINT ( 'NONE',  ( 29.13824727379464008, -291.0908401482650447, -235.5301247027963711 ) ) ;
#2246=ORIENTED_EDGE ( 'NONE', *, *, #76301, .T. ) ;
#2248=CARTESIAN_POINT ( 'NONE',  ( -80.44886470512516041, -289.1615874664133798, -329.4135744628986799 ) ) ;
#2250=CARTESIAN_POINT ( 'NONE',  ( 28.49057261907564254, -287.9757378242036339, -230.7753117105941101 ) ) ;
#2251=CARTESIAN_POINT ( 'NONE',  ( -102.0172624299486870, -286.6233781216988064, -301.5434626090942061 ) ) ;
#2253=CARTESIAN_POINT ( 'NONE',  ( 30.68826836215341558, -293.0711394019737099, -305.9243517995561206 ) ) ;
#2254=CARTESIAN_POINT ( 'NONE',  ( 34.13279988806474563, -283.2150239726330483, -297.6502022334577191 ) ) ;
#2255=CARTESIAN_POINT ( 'NONE',  ( -3.623269331515478253, -282.4274979234524494, -335.1212998712824742 ) ) ;
#2256=CARTESIAN_POINT ( 'NONE',  ( -73.94673581903742843, -273.7467471864824233, -202.5591599092967101 ) ) ;
#2257=CARTESIAN_POINT ( 'NONE',  ( 33.37693755792928840, -277.1305385795566849, -290.4101538631343828 ) ) ;
#2258=CARTESIAN_POINT ( 'NONE',  ( -4.077959936533853025, -290.5130121382752577, -203.5234506636695357 ) ) ;
#2260=CARTESIAN_POINT ( 'NONE',  ( -27.22032104452931733, -272.9784339480717676, -197.6140809357097794 ) ) ;
#2263=CARTESIAN_POINT ( 'NONE',  ( -65.66330152257987152, -287.5991558815953226, -201.4643838546886911 ) ) ;
#2264=CARTESIAN_POINT ( 'NONE',  ( -105.6760030247050395, -297.1803814325327835, -305.2906364265959951 ) ) ;
#2265=CARTESIAN_POINT ( 'NONE',  ( -67.59744818887935480, -286.2957780997120949, -203.8142744977607208 ) ) ;
#2266=CARTESIAN_POINT ( 'NONE',  ( -111.2173512151290282, -277.3486471424189972, -291.2227667612635855 ) ) ;
#2267=CARTESIAN_POINT ( 'NONE',  ( 39.40103137295275104, -294.2744720669308549, -276.0233666051173032 ) ) ;
#2268=CARTESIAN_POINT ( 'NONE',  ( 36.81942048749449725, -285.4938575322436805, -254.7922843445198282 ) ) ;
#2269=CARTESIAN_POINT ( 'NONE',  ( 24.87169684607839315, -294.4875369327571093, -315.7180509856348181 ) ) ;
#2270=CARTESIAN_POINT ( 'NONE',  ( -90.77755225477530132, -291.6009740928693645, -220.5762030113426704 ) ) ;
#2271=DIRECTION ( 'NONE',  ( 0.000000000000000000, 0.000000000000000000, -1.000000000000000000 ) ) ;
#2272=DIRECTION ( 'NONE',  ( 1.000000000000000000, 0.000000000000000000, 0.000000000000000000 ) ) ;
#2273=CARTESIAN_POINT ( 'NONE',  ( -76.15440596509891691, -208.4761271767464166, -353.6627180100853138 ) ) ;
#2274=CARTESIAN_POINT ( 'NONE',  ( -103.4495602201036490, -286.5733906563336291, -232.1448614068082463 ) ) ;
#2275=CARTESIAN_POINT ( 'NONE',  ( 13.79469577742117181, -273.9094976428776818, -334.5364918783848793 ) ) ;
#2277=CARTESIAN_POINT ( 'NONE',  ( -102.0505166742203471, -283.0036781961101724, -304.9219922368613993 ) ) ;
#2278=CARTESIAN_POINT ( 'NONE',  ( -112.6959718101545320, -278.4164608696051459, -254.5661333235538279 ) ) ;
#2279=CARTESIAN_POINT ( 'NONE',  ( 35.22735075649669767, -283.3165065662468010, -252.0399938651215450 ) ) ;
#2280=CARTESIAN_POINT ( 'NONE',  ( 175.7400943157809934, 241.1710852490582795, -178.6611720099773493 ) ) ;
#2281=CARTESIAN_POINT ( 'NONE',  ( -93.01475989681885892, -282.4069054273312531, -322.7168764665680669 ) ) ;
#2282=CARTESIAN_POINT ( 'NONE',  ( 36.58593835799844385, -285.7066235022497835, -280.7763149029742635 ) ) ;
#2283=CARTESIAN_POINT ( 'NONE',  ( -69.62729786191843573, -275.4921578734091554, -201.8053726309009051 ) ) ;
#2284=CARTESIAN_POINT ( 'NONE',  ( -110.4455981908226079, -297.0298829515062948, -271.4703025446996776 ) ) ;
#2285=CARTESIAN_POINT ( 'NONE',  ( 34.70322114486324239, -292.0467435590864511, -255.8431016554352766 ) ) ;
#2286=CARTESIAN_POINT ( 'NONE',  ( -95.12870360745725407, -278.5160725051208033, -321.0954753319850852 ) ) ;
#2287=CARTESIAN_POINT ( 'NONE',  ( 0.8714263338593288832, -276.5272476975952145, -332.6198467689641234 ) ) ;
#2288=CARTESIAN_POINT ( 'NONE',  ( -110.7452984687751751, -273.9138284787135831, -247.9667738070575069 ) ) ;
#2289=CARTESIAN_POINT ( 'NONE',  ( -35.73183820551313516, -275.9527672792785893, -347.0481797648846509 ) ) ;
#2290=CARTESIAN_POINT ( 'NONE',  ( -56.60324186025278692, -169.1846951021010170, -364.3055494911728829 ) ) ;
#2291=CARTESIAN_POINT ( 'NONE',  ( -95.68291027872491838, -275.9030506399489013, -317.5118654783422585 ) ) ;
#2292=CARTESIAN_POINT ( 'NONE',  ( 15.08767394035932163, -295.7547411620569733, -325.9467908356010071 ) ) ;
#2295=CARTESIAN_POINT ( 'NONE',  ( 151.9709352735115147, -299.5541904835127980, -195.3611179825600175 ) ) ;
#2296=CARTESIAN_POINT ( 'NONE',  ( -110.1782350143009808, -285.5169185262721498, -279.1088324629775457 ) ) ;
#2297=CARTESIAN_POINT ( 'NONE',  ( -47.10368354335948737, -284.9346812822123525, -345.7181195953769475 ) ) ;
#2298=CARTESIAN_POINT ( 'NONE',  ( -52.10142168324821910, -285.2067626783365881, -198.7647264013608606 ) ) ;
#2299=CARTESIAN_POINT ( 'NONE',  ( -110.9680387438430813, -276.8768546226355625, -276.1212530909722318 ) ) ;
#2300=CARTESIAN_POINT ( 'NONE',  ( -105.2335585894003600, -286.0151975573086816, -300.3871239151109194 ) ) ;
#2301=CARTESIAN_POINT ( 'NONE',  ( -77.18055106536478149, -277.9877595503423890, -208.3037345103906546 ) ) ;
#2302=CARTESIAN_POINT ( 'NONE',  ( -37.79794088248138451, -278.1376362845738299, -343.6813172707657600 ) ) ;
#2304=CARTESIAN_POINT ( 'NONE',  ( -100.7743049724189177, -273.5420382400129711, -234.0061868943173806 ) ) ;
#2305=CARTESIAN_POINT ( 'NONE',  ( 10.71403707775604630, -281.4996777104981334, -210.3362354427328853 ) ) ;
#2306=CARTESIAN_POINT ( 'NONE',  ( -17.01428821104827094, -280.8001592551700014, -196.1565141643202423 ) ) ;
#2310=CARTESIAN_POINT ( 'NONE',  ( -0.3404726754234554398, -288.3990524599335004, -204.2311519053499751 ) ) ;
#2311=CARTESIAN_POINT ( 'NONE',  ( -79.81349927328808747, -296.6582700005264996, -210.7897489880191984 ) ) ;
#2314=CARTESIAN_POINT ( 'NONE',  ( -86.44156338526975958, -290.7397834800261194, -211.1099247157329444 ) ) ;
#2315=CARTESIAN_POINT ( 'NONE',  ( 16.50445825212031536, -286.7495665182208882, -320.7477781803256107 ) ) ;
#2317=CARTESIAN_POINT ( 'NONE',  ( -72.65745444598745451, -288.1042941246570877, -334.9225028419774048 ) ) ;
#2318=CARTESIAN_POINT ( 'NONE',  ( -96.09295359081254162, -286.3713954302164097, -226.3677011752311046 ) ) ;
#2319=CARTESIAN_POINT ( 'NONE',  ( -76.78532099673294908, -275.5796475823318019, -334.2117729292891113 ) ) ;
#2320=CARTESIAN_POINT ( 'NONE',  ( 9.717715720091057108, -286.8169561901785869, -330.3602902612408343 ) ) ;
#2321=CARTESIAN_POINT ( 'NONE',  ( 29.62429522301378171, -289.1061269922853967, -236.5889976418591232 ) ) ;
#2322=CARTESIAN_POINT ( 'NONE',  ( -20.92229114266228507, -286.8418832625529262, -343.7659035601654978 ) ) ;
#2324=CARTESIAN_POINT ( 'NONE',  ( 12.08428806789046739, -283.2854833372259122, -324.4025848245134398 ) ) ;
#2325=CARTESIAN_POINT ( 'NONE',  ( -112.5553537023478441, -292.5411397825399717, -271.2335204130772581 ) ) ;
#2328=CARTESIAN_POINT ( 'NONE',  ( -97.11024979582101935, -299.1013985599712441, -224.1121546556895510 ) ) ;
#2330=CARTESIAN_POINT ( 'NONE',  ( 33.91999220654804503, -280.5312872617810172, -253.7969115975176067 ) ) ;
#2331=CARTESIAN_POINT ( 'NONE',  ( 37.01910815044121961, -279.4215622442448534, -260.2030912569527459 ) ) ;
#2332=CARTESIAN_POINT ( 'NONE',  ( -13.84117010841714901, -293.9519134314286362, -343.5176891770710199 ) ) ;
#2333=CARTESIAN_POINT ( 'NONE',  ( -70.81236020727760661, -296.0029299564718031, -204.5735400505934081 ) ) ;
#2334=CARTESIAN_POINT ( 'NONE',  ( -15.99078679757546340, -274.8538637697693616, -341.7275270703441947 ) ) ;
#2335=CARTESIAN_POINT ( 'NONE',  ( -2.897907067329185349, -295.9020067124427555, -335.2831373490424198 ) ) ;
#2337=CARTESIAN_POINT ( 'NONE',  ( -73.64876197396921498, -272.1550520232934787, -203.0683588118110379 ) ) ;
#2338=CARTESIAN_POINT ( 'NONE',  ( -63.93285093123521534, -293.6341073546713005, -341.5431712844045933 ) ) ;
#2339=CARTESIAN_POINT ( 'NONE',  ( -37.56985275435032179, -293.4745510285827095, -196.7596968199149501 ) ) ;
#2341=CARTESIAN_POINT ( 'NONE',  ( 23.07210063998580196, -294.9289462310797489, -311.7144138195880601 ) ) ;
#2343=CARTESIAN_POINT ( 'NONE',  ( -110.2892195143455041, -282.3300111003733832, -289.3085383194310225 ) ) ;
#2344=CARTESIAN_POINT ( 'NONE',  ( 27.15807033942866155, -294.0191603917574525, -304.6565546054134188 ) ) ;
#2346=CARTESIAN_POINT ( 'NONE',  ( -66.57625017306888537, -283.4246095075651510, -341.6097132827006817 ) ) ;
#2347=CARTESIAN_POINT ( 'NONE',  ( 35.21007397252864735, -283.2020155370854013, -249.2066292902416365 ) ) ;
#2348=CARTESIAN_POINT ( 'NONE',  ( -93.90131680918844381, -284.9307287537023399, -218.0646712839107693 ) ) ;
#2349=CARTESIAN_POINT ( 'NONE',  ( -100.4000020614363393, -288.0083156824197204, -310.6560181938254459 ) ) ;
#2351=CARTESIAN_POINT ( 'NONE',  ( 19.25612745805068471, -280.7340573207635543, -321.6184119485980659 ) ) ;
#2352=CARTESIAN_POINT ( 'NONE',  ( 11.47404437362297180, -285.4305280864174961, -215.3539756115959563 ) ) ;
#2353=CARTESIAN_POINT ( 'NONE',  ( 36.84190215760990839, -286.7169291577924923, -289.8106851383240041 ) ) ;
#2354=CARTESIAN_POINT ( 'NONE',  ( 19.46176235605588900, -295.8132373981581509, -317.4759465088477555 ) ) ;
#2355=CARTESIAN_POINT ( 'NONE',  ( -97.24635011782608274, -280.6170286888922760, -222.9265398223296302 ) ) ;
#2356=CARTESIAN_POINT ( 'NONE',  ( -52.97321076489322422, -293.2715185747370583, -344.1305950818194219 ) ) ;
#2357=CARTESIAN_POINT ( 'NONE',  ( -16.91173510106462174, -279.9900987005459569, -200.2561679740749980 ) ) ;
#2358=CARTESIAN_POINT ( 'NONE',  ( 37.76083416989510511, -293.5056996349703127, -253.3135023623635504 ) ) ;
#2359=CARTESIAN_POINT ( 'NONE',  ( -108.8695594198320720, -282.3193183739194865, -294.7143424573694688 ) ) ;
#2360=CARTESIAN_POINT ( 'NONE',  ( -39.86935474058879691, -279.0840375942528340, -345.3312437491790092 ) ) ;
#2361=CARTESIAN_POINT ( 'NONE',  ( -73.42875210752718829, -294.6022849606284240, -334.0881383726343756 ) ) ;
#2362=CARTESIAN_POINT ( 'NONE',  ( -51.40008341153777849, -295.8723580452389115, -196.6375582276594969 ) ) ;
#2365=CARTESIAN_POINT ( 'NONE',  ( -1.191090837588199225, -282.5142281842524312, -205.0543017072447185 ) ) ;
#2366=CARTESIAN_POINT ( 'NONE',  ( -45.10350010521774777, -294.6606065751674350, -343.0597130516309221 ) ) ;
#2368=CARTESIAN_POINT ( 'NONE',  ( -37.37352853689063181, -274.5523547857346784, -345.3611179825600175 ) ) ;
#2369=CARTESIAN_POINT ( 'NONE',  ( 11.69052944090781310, -273.9097949304809276, -211.1311788300132264 ) ) ;
#2370=CARTESIAN_POINT ( 'NONE',  ( -26.19972767792013713, -290.2283118574376886, -346.0522979289643786 ) ) ;
#2371=CARTESIAN_POINT ( 'NONE',  ( -106.9527405965465476, -290.0920538385502709, -292.5124797387500166 ) ) ;
#2372=CARTESIAN_POINT ( 'NONE',  ( -30.21441684358461544, -281.6639377239478677, -196.9624178316807956 ) ) ;
#2373=CARTESIAN_POINT ( 'NONE',  ( -109.9202075428785577, -274.3303380581464808, -256.7157215857342294 ) ) ;
#2374=CARTESIAN_POINT ( 'NONE',  ( 7.396438086658410072, -279.4723336308808257, -212.1106403080696907 ) ) ;
#2376=CARTESIAN_POINT ( 'NONE',  ( 11.78732464390185797, -274.5458451004375320, -211.0015375460011740 ) ) ;
#2377=CARTESIAN_POINT ( 'NONE',  ( -36.20825719148006527, -293.9865892983897311, -195.9170205862630496 ) ) ;
#2379=EDGE_CURVE ( 'NONE', #14296, #31036, #74788, .T. ) ;
#2381=CARTESIAN_POINT ( 'NONE',  ( -36.37002147508545846, -290.2038029420513681, -194.5897215437361751 ) ) ;
#2382=CARTESIAN_POINT ( 'NONE',  ( -36.47883191666217328, -297.7299650106613740, -197.3400242297411182 ) ) ;
#2385=CARTESIAN_POINT ( 'NONE',  ( -113.5578456738071935, -292.0253799048121550, -274.0768829384814467 ) ) ;
#2386=CARTESIAN_POINT ( 'NONE',  ( -19.11405058567862625, -294.7662352645559736, -190.3538533559490702 ) ) ;
#2387=CARTESIAN_POINT ( 'NONE',  ( 30.46055287969270253, -289.1351492837338242, -238.6927913698075372 ) ) ;
#2388=CARTESIAN_POINT ( 'NONE',  ( -10.62266284991046028, -274.7026527243753549, -340.2619153569320929 ) ) ;
#2389=CARTESIAN_POINT ( 'NONE',  ( 20.96851465639591439, -276.8315246912528096, -224.0672715805402504 ) ) ;
#2390=CARTESIAN_POINT ( 'NONE',  ( 3.041837134920090335, -290.6784192119872614, -207.7661812040237805 ) ) ;
#2391=CARTESIAN_POINT ( 'NONE',  ( -56.27131836490882932, -281.6713580191880055, -196.9450497220784086 ) ) ;
#2394=CARTESIAN_POINT ( 'NONE',  ( -53.72056482496905261, -282.6163832278657537, -341.6567004821625915 ) ) ;
#2395=CARTESIAN_POINT ( 'NONE',  ( -77.64072628188118586, -278.6589829938239973, -335.6721994885797358 ) ) ;
#2396=CARTESIAN_POINT ( 'NONE',  ( 17.53107308459359714, -281.0844438218102823, -323.8876904598456008 ) ) ;
#2397=CARTESIAN_POINT ( 'NONE',  ( -100.2657439814591385, -278.9103520919917401, -314.3313911027744894 ) ) ;
#2398=CARTESIAN_POINT ( 'NONE',  ( -2.888072313469212116, -276.0192265579439663, -202.2609024276526668 ) ) ;
#2399=CARTESIAN_POINT ( 'NONE',  ( 27.36219212280431989, -284.4805209788416391, -301.4846348637938149 ) ) ;
#2400=ORIENTED_EDGE ( 'NONE', *, *, #55197, .T. ) ;
#2401=CARTESIAN_POINT ( 'NONE',  ( -112.3848973411877950, -298.5374536137122732, -271.5187285978493037 ) ) ;
#2402=CARTESIAN_POINT ( 'NONE',  ( -86.92839002084259903, -290.8411630607247957, -324.4242874364562681 ) ) ;
#2403=CARTESIAN_POINT ( 'NONE',  ( -13.27849275885741065, -274.7583160877609316, -341.0752561779326015 ) ) ;
#2404=CARTESIAN_POINT ( 'NONE',  ( -70.18057860147415283, -291.2389563376514161, -338.8997289832494744 ) ) ;
#2405=CARTESIAN_POINT ( 'NONE',  ( -94.36521346548927625, -290.5465004580488539, -224.6005297093131219 ) ) ;
#2406=CARTESIAN_POINT ( 'NONE',  ( 37.31863131032162784, -286.8271222588363116, -251.7772052354250718 ) ) ;
#2408=CARTESIAN_POINT ( 'NONE',  ( -110.2077907440444022, -283.1057778829976996, -258.5776496901708583 ) ) ;
#2409=CARTESIAN_POINT ( 'NONE',  ( -106.2509406892953052, -292.0475346752432984, -298.1102357068517676 ) ) ;
#2410=CARTESIAN_POINT ( 'NONE',  ( -62.78424581810185146, -284.1948704720394403, -201.1446866725465838 ) ) ;
#2411=CARTESIAN_POINT ( 'NONE',  ( 0.6405716419054025002, -281.8848009400309707, -207.3848841765032773 ) ) ;
#2412=CARTESIAN_POINT ( 'NONE',  ( 31.48180083919579886, -288.9330326451807878, -304.4831849100746126 ) ) ;
#2413=CARTESIAN_POINT ( 'NONE',  ( -91.34652890947378978, -279.7495179408469426, -221.1527151429708056 ) ) ;
#2414=CARTESIAN_POINT ( 'NONE',  ( 34.09810750059581608, -291.9933715860795473, -242.5673455710627593 ) ) ;
#2415=CARTESIAN_POINT ( 'NONE',  ( 38.51723649147143647, -288.5123174863997519, -282.9151757114605061 ) ) ;
#2416=CARTESIAN_POINT ( 'NONE',  ( -69.77261671130307263, -286.1288604391023114, -200.5774111389115149 ) ) ;
#2417=CARTESIAN_POINT ( 'NONE',  ( -84.86017187945472529, -283.8959858414048654, -325.7776754983261753 ) ) ;
#2420=CARTESIAN_POINT ( 'NONE',  ( 33.30238579561800805, -295.0583696151126105, -242.8352620235359609 ) ) ;
#2421=CARTESIAN_POINT ( 'NONE',  ( 17.19816457336363058, -292.9790586830068833, -324.0899834076009256 ) ) ;
#2422=CARTESIAN_POINT ( 'NONE',  ( -16.32477394961795980, -275.8326082407812123, -340.5691043169587147 ) ) ;
#2423=CARTESIAN_POINT ( 'NONE',  ( -70.67734101756153109, -296.9725667447256683, -201.0643082889385767 ) ) ;
#2424=CARTESIAN_POINT ( 'NONE',  ( 35.59671247223678847, -291.8945387362592214, -259.8399146305260388 ) ) ;
#2425=CARTESIAN_POINT ( 'NONE',  ( -110.8131974872760139, -294.6703414406898673, -279.7119362418612241 ) ) ;
#2426=CARTESIAN_POINT ( 'NONE',  ( -4.670041263478490023, -293.6974645934221826, -204.6227457080949250 ) ) ;
#2427=CARTESIAN_POINT ( 'NONE',  ( 23.59055957170356521, -294.0681241304459377, -229.5997907031644161 ) ) ;
#2429=CARTESIAN_POINT ( 'NONE',  ( -22.48541094444601995, -292.8622030144426844, -344.0450313913269724 ) ) ;
#2430=CARTESIAN_POINT ( 'NONE',  ( -104.9446028033678431, -298.9813624462061057, -237.7643205647046614 ) ) ;
#2431=CARTESIAN_POINT ( 'NONE',  ( 27.24360732475430780, -288.9638346358789249, -304.9965575090857897 ) ) ;
#2432=CARTESIAN_POINT ( 'NONE',  ( -64.47869382042421194, -279.3843633652002154, -340.7154844104159110 ) ) ;
#2433=CARTESIAN_POINT ( 'NONE',  ( 3.277872121411345763, -275.3145317421886489, -335.3701372609937721 ) ) ;
#2435=CARTESIAN_POINT ( 'NONE',  ( 1.151591253278470894, -273.9005858307074277, -203.7757440722843967 ) ) ;
#2436=CARTESIAN_POINT ( 'NONE',  ( 25.32983365565038980, -280.1780890191662934, -310.6253857454715899 ) ) ;
#2437=CARTESIAN_POINT ( 'NONE',  ( -25.91030507356118662, -275.3087558394569214, -345.6987820090255354 ) ) ;
#2439=CARTESIAN_POINT ( 'NONE',  ( -110.7350194627203450, -295.1867942690556674, -274.1904983298594516 ) ) ;
#2440=CARTESIAN_POINT ( 'NONE',  ( -65.99069756724364311, -275.6774747864053552, -201.0348621853013356 ) ) ;
#2441=CARTESIAN_POINT ( 'NONE',  ( -92.99677433997791809, -273.8769465895456960, -222.9455333364743126 ) ) ;
#2443=CARTESIAN_POINT ( 'NONE',  ( -106.2380124564062953, -288.1727745790136623, -301.0133967033503950 ) ) ;
#2444=CARTESIAN_POINT ( 'NONE',  ( -32.68891170524955925, -273.9457094342653818, -197.4970195534421293 ) ) ;
#2445=CARTESIAN_POINT ( 'NONE',  ( -9.563331133520202698, -288.6990254255125024, -342.1758951248863809 ) ) ;
#2446=CARTESIAN_POINT ( 'NONE',  ( -15.43315215435428911, -300.3050012637568784, -194.9985599119324604 ) ) ;
#2447=CARTESIAN_POINT ( 'NONE',  ( -93.58499416087970246, -293.8646530689550218, -319.7242652163323555 ) ) ;
#2448=CARTESIAN_POINT ( 'NONE',  ( -41.57049742590108110, -282.3011711864564859, -347.1354049258234227 ) ) ;
#2450=CARTESIAN_POINT ( 'NONE',  ( 32.33756184536254352, -279.9149438931633540, -298.2448987394334949 ) ) ;
#2454=CARTESIAN_POINT ( 'NONE',  ( -108.8106150073328564, -289.5670728927869959, -253.5933460248497227 ) ) ;
#2455=CARTESIAN_POINT ( 'NONE',  ( -102.8725561325814226, -282.2230593162726677, -305.3499860189297692 ) ) ;
#2458=CARTESIAN_POINT ( 'NONE',  ( -107.5747994095082873, -288.8953773185871228, -243.9020588889401893 ) ) ;
#2459=CARTESIAN_POINT ( 'NONE',  ( -59.70429240495381151, -275.2774344503241650, -200.0892990232544548 ) ) ;
#2460=CARTESIAN_POINT ( 'NONE',  ( -81.32097392682602788, -284.8402280689018085, -333.1459105784276744 ) ) ;
#2461=CARTESIAN_POINT ( 'NONE',  ( -13.49336395985828752, -272.4392708445743665, -198.6633421562725630 ) ) ;
#2462=CARTESIAN_POINT ( 'NONE',  ( -10.74997186824332474, -286.4088293835263812, -202.3631822162128344 ) ) ;
#2463=CARTESIAN_POINT ( 'NONE',  ( 35.69318083708846245, -277.1007374102973699, -279.7839234860754232 ) ) ;
#2464=CARTESIAN_POINT ( 'NONE',  ( 30.43146551669902422, -276.7249088396201273, -298.0531741480480150 ) ) ;
#2465=CARTESIAN_POINT ( 'NONE',  ( -34.52782412456014782, -285.0169364489924533, -345.3083177512349948 ) ) ;
#2468=CARTESIAN_POINT ( 'NONE',  ( -41.94768288338276108, -294.9418706406960382, -347.2756277286085265 ) ) ;
#2469=CARTESIAN_POINT ( 'NONE',  ( 32.50494542338549309, -289.1867028367436205, -243.8848862199949963 ) ) ;
#2471=CARTESIAN_POINT ( 'NONE',  ( 40.64545035920995986, -291.2666405000203440, -288.1938231032136741 ) ) ;
#2472=CARTESIAN_POINT ( 'NONE',  ( -112.1857616634828645, -277.2624241539681407, -287.0901037333476893 ) ) ;
#2473=CARTESIAN_POINT ( 'NONE',  ( -103.9011893556237141, -289.4380373701298481, -233.2629400291850175 ) ) ;
#2474=CARTESIAN_POINT ( 'NONE',  ( -110.6864656399369693, -286.1724318225008687, -262.6970049916134258 ) ) ;
#2475=CARTESIAN_POINT ( 'NONE',  ( -95.60222064919906870, -280.9472530154350807, -224.6933035624708168 ) ) ;
#2476=CARTESIAN_POINT ( 'NONE',  ( -54.84737931417252099, -287.2566344071678941, -195.9826433577420630 ) ) ;
#2477=CARTESIAN_POINT ( 'NONE',  ( -12.85290433956945577, -284.7341782101797207, -341.3055452751005987 ) ) ;
#2478=CARTESIAN_POINT ( 'NONE',  ( -42.80405109958635990, -277.2859728771105097, -347.1671250807937668 ) ) ;
#2479=CARTESIAN_POINT ( 'NONE',  ( -102.2967516304183846, -271.0499318740187960, -233.0969194531548396 ) ) ;
#2480=CARTESIAN_POINT ( 'NONE',  ( -19.75416020125787142, -280.1054263353923375, -195.3418325556406216 ) ) ;
#2481=CARTESIAN_POINT ( 'NONE',  ( -109.2326051827405280, -298.7230397365784142, -250.9984197659080394 ) ) ;
#2483=CARTESIAN_POINT ( 'NONE',  ( -85.28047601435908120, -280.1948066931273047, -330.5268031993605859 ) ) ;
#2484=CARTESIAN_POINT ( 'NONE',  ( -31.99397031523169943, -296.2580116381537323, -194.5979839244863285 ) ) ;
#2486=CARTESIAN_POINT ( 'NONE',  ( -72.87741659627590707, -277.0441251465967412, -334.2128157899669532 ) ) ;
#2487=CARTESIAN_POINT ( 'NONE',  ( -29.89284046659686922, -275.3495337395068532, -194.1212123687265603 ) ) ;
#2488=CARTESIAN_POINT ( 'NONE',  ( 39.17812565146557091, -280.5340444180471877, -264.2344161684337678 ) ) ;
#2489=CARTESIAN_POINT ( 'NONE',  ( 29.14777769934636709, -289.7466609382010461, -302.8745513465544263 ) ) ;
#2490=CARTESIAN_POINT ( 'NONE',  ( -111.6041093367672801, -298.2936890885879961, -252.8168216423337640 ) ) ;
#2491=CARTESIAN_POINT ( 'NONE',  ( -90.42579470457449986, -296.9883760940584239, -325.6617309611877999 ) ) ;
#2492=CARTESIAN_POINT ( 'NONE',  ( 14.14656434473762658, -294.7774907196733807, -216.0565413230712863 ) ) ;
#2493=CARTESIAN_POINT ( 'NONE',  ( 23.28257652777596221, -280.1509791272385428, -314.2547421445567579 ) ) ;
#2494=CARTESIAN_POINT ( 'NONE',  ( 37.00532661597684836, -283.5204280807112127, -274.0805009427418781 ) ) ;
#2495=CARTESIAN_POINT ( 'NONE',  ( -103.8072740394163418, -295.0795299535373033, -236.7256545338261731 ) ) ;
#2496=CARTESIAN_POINT ( 'NONE',  ( -15.77377628421712252, -287.6869322676240017, -340.4787815142049112 ) ) ;
#2497=CARTESIAN_POINT ( 'NONE',  ( 7.406912897105986104, -59.46167575493636548, -354.1292707482897413 ) ) ;
#2499=CARTESIAN_POINT ( 'NONE',  ( 18.20392823275637539, -286.8490286691834399, -322.8329148141617679 ) ) ;
#2500=CARTESIAN_POINT ( 'NONE',  ( 2.462092760079154452, -286.2687590341921577, -209.1422846185902529 ) ) ;
#2502=CARTESIAN_POINT ( 'NONE',  ( -52.84164399697896641, -284.3258424455721070, -345.5236060886878136 ) ) ;
#2503=CARTESIAN_POINT ( 'NONE',  ( -0.5392800613394916898, -274.8890477393947549, -207.2777563747063425 ) ) ;
#2504=CARTESIAN_POINT ( 'NONE',  ( -70.75058481462328075, -290.5420937758617015, -201.3296835817472470 ) ) ;
#2505=CARTESIAN_POINT ( 'NONE',  ( 39.17755701731379503, -282.3054800828855377, -278.4994843734720575 ) ) ;
#2506=CARTESIAN_POINT ( 'NONE',  ( 37.57030566641581260, -282.8889962433487426, -255.8387510213572114 ) ) ;
#2507=CARTESIAN_POINT ( 'NONE',  ( 37.65593532437416258, -281.6677040430466832, -252.9510138777561394 ) ) ;
#2509=CARTESIAN_POINT ( 'NONE',  ( -22.19440711724928050, -280.2514718432173595, -198.8980604804226289 ) ) ;
#2510=CARTESIAN_POINT ( 'NONE',  ( -6.998514795304330072, -292.1237833571632336, -333.4427485647536855 ) ) ;
#2511=CARTESIAN_POINT ( 'NONE',  ( -12.44406248820926209, -91.84162952613797870, -360.1898987475070157 ) ) ;
#2513=CARTESIAN_POINT ( 'NONE',  ( 30.74374590970317911, -277.1423916912688696, -239.1810597560504732 ) ) ;
#2514=CARTESIAN_POINT ( 'NONE',  ( 201.3707903610551284, 293.7126099848096032, -83.13998816544706472 ) ) ;
#2515=CARTESIAN_POINT ( 'NONE',  ( 29.26011548929556128, -279.1233857181673557, -236.5411674088905727 ) ) ;
#2516=CARTESIAN_POINT ( 'NONE',  ( -96.96107154359567915, -296.4906081440020102, -228.0595433029909884 ) ) ;
#2517=CARTESIAN_POINT ( 'NONE',  ( 39.44027207793104850, -293.1308958315894415, -276.0408537448790867 ) ) ;
#2518=CARTESIAN_POINT ( 'NONE',  ( -87.90885014101696981, -230.0150033563139402, -344.6602624353737951 ) ) ;
#2519=CARTESIAN_POINT ( 'NONE',  ( -113.0537791265368242, -271.3799681904797581, -259.0012581418058630 ) ) ;
#2520=CARTESIAN_POINT ( 'NONE',  ( -50.91841670740115688, -287.6282379403374421, -342.9537902857447875 ) ) ;
#2521=CARTESIAN_POINT ( 'NONE',  ( -4.982016089098304512, -296.4819271545327979, -337.1862143980148971 ) ) ;
#2522=CARTESIAN_POINT ( 'NONE',  ( 19.02931575992503355, -288.2022787021525119, -223.1869628898460292 ) ) ;
#2524=CARTESIAN_POINT ( 'NONE',  ( 39.26821225858289921, -294.5642641755329691, -276.0098559517900298 ) ) ;
#2525=CARTESIAN_POINT ( 'NONE',  ( -95.00949098850031760, -285.6762450448375716, -225.4808599488853531 ) ) ;
#2526=CARTESIAN_POINT ( 'NONE',  ( -20.60231402624690134, -297.0522746590115162, -193.7615258097368383 ) ) ;
#2527=CARTESIAN_POINT ( 'NONE',  ( 27.90981592257615418, -293.8219320403491110, -229.6847659620191280 ) ) ;
#2528=CARTESIAN_POINT ( 'NONE',  ( 13.23330608872579361, -293.2297999278542875, -212.3809864784209367 ) ) ;
#2529=CARTESIAN_POINT ( 'NONE',  ( -37.26588755854434254, -289.2178574890489244, -343.3610786469021718 ) ) ;
#2532=CARTESIAN_POINT ( 'NONE',  ( -112.9026085236913275, -274.5078588213003172, -267.5716711293979415 ) ) ;
#2533=CARTESIAN_POINT ( 'NONE',  ( -43.99290773345275340, -272.7649013582303041, -193.9944547808171933 ) ) ;
#2534=CARTESIAN_POINT ( 'NONE',  ( 22.77107744012160850, -281.1920887869873127, -312.1924748982626738 ) ) ;
#2537=CARTESIAN_POINT ( 'NONE',  ( -71.54912814171433411, -276.9996013626940794, -339.2768547356664044 ) ) ;
#2538=CARTESIAN_POINT ( 'NONE',  ( -107.0554866604049522, -271.2705947266883868, -246.1448345789588643 ) ) ;
#2539=CARTESIAN_POINT ( 'NONE',  ( -86.31654927378168907, -281.2242287095804159, -214.5728608944492635 ) ) ;
#2540=CARTESIAN_POINT ( 'NONE',  ( -29.60790894028053089, -275.0929057533552395, -344.2441374449350633 ) ) ;
#2541=CARTESIAN_POINT ( 'NONE',  ( -110.6373970823285475, -297.7066383063740318, -274.2174519674525186 ) ) ;
#2542=CARTESIAN_POINT ( 'NONE',  ( -64.66767662082524737, -274.6276639750179811, -202.4012952673230359 ) ) ;
#2543=CARTESIAN_POINT ( 'NONE',  ( -109.1516566367420751, -274.6296933770493638, -245.5155115500938621 ) ) ;
#2544=CARTESIAN_POINT ( 'NONE',  ( -31.36483227772994553, -272.1473641846681062, -195.2303203988417977 ) ) ;
#2545=CARTESIAN_POINT ( 'NONE',  ( -0.6996809299530281079, -295.2033419772033653, -333.6743699023965064 ) ) ;
#2546=CARTESIAN_POINT ( 'NONE',  ( 33.88304251360246155, -291.8845381301766793, -251.8567683817265959 ) ) ;
#2548=CARTESIAN_POINT ( 'NONE',  ( -37.12084208011064135, -277.5417658976462576, -347.3123111203240114 ) ) ;
#2549=CARTESIAN_POINT ( 'NONE',  ( -106.3070804325457033, -273.0371183426586299, -246.4283721317634388 ) ) ;
#2550=CARTESIAN_POINT ( 'NONE',  ( -24.63210283262489853, -281.5781880969284430, -345.8586685824480469 ) ) ;
#2551=CARTESIAN_POINT ( 'NONE',  ( 0.8601589686108198629, -296.5439030361696382, -335.0963200612210358 ) ) ;
#2553=CARTESIAN_POINT ( 'NONE',  ( -99.17296782236479658, -283.2089455778507272, -309.5647525014836674 ) ) ;
#2554=CARTESIAN_POINT ( 'NONE',  ( -92.11352308361404084, -281.8321099972962998, -321.8588820916905320 ) ) ;
#2555=CARTESIAN_POINT ( 'NONE',  ( 34.46425203079156319, -274.3383407293333676, -286.5205346050232720 ) ) ;
#2556=CARTESIAN_POINT ( 'NONE',  ( 37.70456885433146965, -283.5635385328668008, -271.2350607696074007 ) ) ;
#2557=CARTESIAN_POINT ( 'NONE',  ( 114.7448031289451222, -299.5541904835127980, -195.3611179825600175 ) ) ;
#2559=CARTESIAN_POINT ( 'NONE',  ( -24.27651914122143140, -272.6160209731764894, -195.2359364707425868 ) ) ;
#2560=CARTESIAN_POINT ( 'NONE',  ( -111.1996555297763507, -280.7321098390859220, -256.3268153080034608 ) ) ;
#2561=CARTESIAN_POINT ( 'NONE',  ( 114.7448031289451222, -299.5541904835127980, -195.3611179825600175 ) ) ;
#2562=CARTESIAN_POINT ( 'NONE',  ( 1.970543960950341456, -288.4941262155559230, -205.8331266759901439 ) ) ;
#2564=CARTESIAN_POINT ( 'NONE',  ( -101.6889802861403069, -289.0689421451108387, -231.7330867662568323 ) ) ;
#2565=CARTESIAN_POINT ( 'NONE',  ( 82.12944418934898749, -301.0792019753940849, -196.6542615346262153 ) ) ;
#2566=CARTESIAN_POINT ( 'NONE',  ( -94.26015771298604307, -294.6945015618919115, -316.7211354578644773 ) ) ;
#2567=CARTESIAN_POINT ( 'NONE',  ( -96.77117493611734744, -288.0774781237683442, -314.8683269722934597 ) ) ;
#2568=CARTESIAN_POINT ( 'NONE',  ( -109.0101294763935016, -268.7602059993127455, -295.2240039188629339 ) ) ;
#2569=CARTESIAN_POINT ( 'NONE',  ( -58.44376093788498139, -295.7791764765509015, -198.3909597514329732 ) ) ;
#2570=CARTESIAN_POINT ( 'NONE',  ( 18.12740474629692500, -286.7541943026544686, -322.7623217568016685 ) ) ;
#2571=CARTESIAN_POINT ( 'NONE',  ( 31.08381006476750485, -283.5184984801657038, -298.0087212848238778 ) ) ;
#2572=CARTESIAN_POINT ( 'NONE',  ( -67.50005802522657916, -281.6822348504491060, -340.1067089858914869 ) ) ;
#2574=CARTESIAN_POINT ( 'NONE',  ( -38.89757915434391577, -292.0320934581004622, -197.3777004107880089 ) ) ;
#2575=CARTESIAN_POINT ( 'NONE',  ( 35.06847423779945672, -283.1500458241283695, -283.5520949548027829 ) ) ;
#2576=CARTESIAN_POINT ( 'NONE',  ( -10.90790624518023755, -283.5014575384147975, -338.6339987839949686 ) ) ;
#2577=CARTESIAN_POINT ( 'NONE',  ( -40.24949435402463394, -291.0683929303470450, -345.6730011116519563 ) ) ;
#2578=CARTESIAN_POINT ( 'NONE',  ( 53.58540442190474096, -299.3278094806844365, -193.3585760710489296 ) ) ;
#2579=CARTESIAN_POINT ( 'NONE',  ( -71.28197762215567934, -287.5766138327124963, -337.8694268440394239 ) ) ;
#2580=CARTESIAN_POINT ( 'NONE',  ( 39.55433251004694739, -275.4906040140362506, -265.4397775109711688 ) ) ;
#2581=CARTESIAN_POINT ( 'NONE',  ( -80.50183842382482169, -293.4442452339447414, -209.3957841586187669 ) ) ;
#2583=CARTESIAN_POINT ( 'NONE',  ( -37.30987171927208124, -285.5519495502701943, -345.3611179825600175 ) ) ;
#2584=CARTESIAN_POINT ( 'NONE',  ( -112.4026414192340582, -276.5009297402772859, -274.3465309319217909 ) ) ;
#2586=CARTESIAN_POINT ( 'NONE',  ( -36.88214745873715117, -296.4576934405298516, -194.1612352087267084 ) ) ;
#2587=CARTESIAN_POINT ( 'NONE',  ( -30.75565191114682051, -293.7369253260489472, -196.8555781642556894 ) ) ;
#2588=CARTESIAN_POINT ( 'NONE',  ( -83.24816674809036954, -272.7523357296409472, -213.4709695358284307 ) ) ;
#2589=CARTESIAN_POINT ( 'NONE',  ( -98.67710828325509453, -291.5102581345895487, -311.2335064567484437 ) ) ;
#2590=CARTESIAN_POINT ( 'NONE',  ( -33.50806778203349268, -293.0428103764843399, -197.2136983412937639 ) ) ;
#2591=CARTESIAN_POINT ( 'NONE',  ( -106.5199209340004671, -286.6587904436104282, -244.0486156681365060 ) ) ;
#2592=CARTESIAN_POINT ( 'NONE',  ( -96.13719915801695493, -292.6388694983503456, -221.5382730703051664 ) ) ;
#2593=CARTESIAN_POINT ( 'NONE',  ( -97.96781482763074678, -292.4942450918965164, -223.6733031492414057 ) ) ;
#2594=CARTESIAN_POINT ( 'NONE',  ( -47.79513500865209608, -295.0219697449707041, -342.6600672993502030 ) ) ;
#2595=CARTESIAN_POINT ( 'NONE',  ( 29.42735459738318937, -289.0992210889988883, -236.0868579360104320 ) ) ;
#2596=CARTESIAN_POINT ( 'NONE',  ( 35.32698080185477352, -281.3958981561121959, -244.7408750858148210 ) ) ;
#2597=CARTESIAN_POINT ( 'NONE',  ( -37.57814693287620145, -296.1290649032766282, -194.8014839469518336 ) ) ;
#2598=CARTESIAN_POINT ( 'NONE',  ( -114.1516837733771297, -284.4619489567068058, -264.2461254498870176 ) ) ;
#2599=CARTESIAN_POINT ( 'NONE',  ( 29.31909782075390680, -277.0862027302344472, -236.7726554332141404 ) ) ;
#2600=CARTESIAN_POINT ( 'NONE',  ( -30.47895674286609236, -284.9356444255347469, -197.2345115044694808 ) ) ;
#2601=CARTESIAN_POINT ( 'NONE',  ( 33.18288295963861856, -285.8846397858544037, -296.0323353182214987 ) ) ;
#2602=CARTESIAN_POINT ( 'NONE',  ( -59.32954263216747393, -275.4734228370343203, -342.8651886295908184 ) ) ;
#2604=CARTESIAN_POINT ( 'NONE',  ( -32.14757809627998597, -282.4925156143311256, -343.2377914661568639 ) ) ;
#2605=CARTESIAN_POINT ( 'NONE',  ( -98.26991588888164131, -280.3795870676837012, -223.9095691879708738 ) ) ;
#2606=CARTESIAN_POINT ( 'NONE',  ( 26.94727416595988601, -286.0581247976591044, -228.4117676061393354 ) ) ;
#2607=CARTESIAN_POINT ( 'NONE',  ( -12.64933399778398559, -296.4869600891081518, -340.1880473644476979 ) ) ;
#2608=CARTESIAN_POINT ( 'NONE',  ( 10.04466864528783354, -278.0119495135026000, -330.1023947800194946 ) ) ;
#2610=CARTESIAN_POINT ( 'NONE',  ( 37.42732865843625234, -277.0721754823205174, -286.6362892232604054 ) ) ;
#2611=CARTESIAN_POINT ( 'NONE',  ( -76.35761310689036918, -277.4227705535585642, -332.1195040930644495 ) ) ;
#2613=CARTESIAN_POINT ( 'NONE',  ( -111.9865001276049412, -274.5317257338260788, -270.3862691793228805 ) ) ;
#2614=CARTESIAN_POINT ( 'NONE',  ( 34.80335845759631752, -285.2957740370831630, -250.4835187737770639 ) ) ;
#2615=CARTESIAN_POINT ( 'NONE',  ( -95.76443986161672228, -291.4867524763847655, -319.3019374003989697 ) ) ;
#2616=CARTESIAN_POINT ( 'NONE',  ( -37.00789244456584015, -293.9681698002687540, -343.6819476778110811 ) ) ;
#2618=CARTESIAN_POINT ( 'NONE',  ( -3.622721304443028867, -292.1768241087224283, -205.5913877535546703 ) ) ;
#2620=CARTESIAN_POINT ( 'NONE',  ( -99.61121219932368831, -291.0357986268933246, -315.1496747525023352 ) ) ;
#2621=CARTESIAN_POINT ( 'NONE',  ( -79.11990784704468638, -280.1231263425738689, -210.3738357661613350 ) ) ;
#2622=CARTESIAN_POINT ( 'NONE',  ( -112.5827296610251267, -295.6596985770443098, -255.4518117481867137 ) ) ;
#2623=CARTESIAN_POINT ( 'NONE',  ( 33.95095192629591452, -288.5715524420124893, -299.3243443023405916 ) ) ;
#2624=CARTESIAN_POINT ( 'NONE',  ( -5.631326695201923194, -288.9796607209196964, -340.5052304109456713 ) ) ;
#2625=CARTESIAN_POINT ( 'NONE',  ( -64.05915791857650277, -283.7438051644921302, -338.3189353106994872 ) ) ;
#2626=CARTESIAN_POINT ( 'NONE',  ( -114.0438014765299215, -273.4268578961535354, -284.1485094271377534 ) ) ;
#2627=CARTESIAN_POINT ( 'NONE',  ( -112.9922304011642495, -269.2718471480555991, -295.9038691064662316 ) ) ;
#2628=CARTESIAN_POINT ( 'NONE',  ( -70.50382606843994893, -195.7257949056034931, -356.6408436669652247 ) ) ;
#2629=CARTESIAN_POINT ( 'NONE',  ( 16.64341557793552084, -275.4562902256799362, -319.7580243250421859 ) ) ;
#2630=CARTESIAN_POINT ( 'NONE',  ( -109.4335942592762052, -277.6472334744765931, -257.0575517376553307 ) ) ;
#2631=CARTESIAN_POINT ( 'NONE',  ( -78.82658720551361853, -273.1760358027513007, -205.5170863709533364 ) ) ;
#2632=CARTESIAN_POINT ( 'NONE',  ( -109.1074448185741090, -269.9587199336866661, -295.5484694788251545 ) ) ;
#2633=CARTESIAN_POINT ( 'NONE',  ( -90.99521459593580630, -276.4792331045256901, -324.9752046622032822 ) ) ;
#2635=CARTESIAN_POINT ( 'NONE',  ( -106.6316394200870548, -291.3519773509669903, -247.1901716369108328 ) ) ;
#2636=CARTESIAN_POINT ( 'NONE',  ( -78.12543314815535211, -298.3213695714580354, -205.2393402026673357 ) ) ;
#2637=CARTESIAN_POINT ( 'NONE',  ( 32.77912136034463231, -286.5286944658053585, -292.5375017262568917 ) ) ;
#2638=CARTESIAN_POINT ( 'NONE',  ( -35.48006003109107809, -298.5672192782942602, -193.4225051656221410 ) ) ;
#2639=CARTESIAN_POINT ( 'NONE',  ( -18.21845782763830357, -294.9654075725447910, -340.8118213743876481 ) ) ;
#2642=CARTESIAN_POINT ( 'NONE',  ( -70.90874729217547667, -279.4117121779906370, -338.0557820761433163 ) ) ;
#2643=CARTESIAN_POINT ( 'NONE',  ( 4.506962441440763634, -282.0117511107029600, -334.9858077310677800 ) ) ;
#2644=CARTESIAN_POINT ( 'NONE',  ( -93.33516388618359372, -280.3016055325900879, -223.0241738132965281 ) ) ;
#2645=CARTESIAN_POINT ( 'NONE',  ( -111.7961672262611614, -280.1190645538988520, -285.6077653152621565 ) ) ;
#2646=CARTESIAN_POINT ( 'NONE',  ( -109.2067726620527708, -271.2452017205010293, -254.0479605788654851 ) ) ;
#2648=CARTESIAN_POINT ( 'NONE',  ( -49.14399963614311417, -280.0642257073692463, -198.3215057486694377 ) ) ;
#2649=CARTESIAN_POINT ( 'NONE',  ( -104.0943289132476224, -273.8514872881061706, -232.1984954337163742 ) ) ;
#2650=CARTESIAN_POINT ( 'NONE',  ( -66.77485199109769098, -275.6666780879847352, -201.3778575332219134 ) ) ;
#2651=CARTESIAN_POINT ( 'NONE',  ( 14.47020840095260574, -274.9153759317688355, -326.5947789362264189 ) ) ;
#2653=CARTESIAN_POINT ( 'NONE',  ( -109.8587725886749098, -289.8817878628083804, -260.2967924051071122 ) ) ;
#2654=CARTESIAN_POINT ( 'NONE',  ( -73.55766334611128343, -284.9334191828816074, -202.4661896362791254 ) ) ;
#2655=CARTESIAN_POINT ( 'NONE',  ( 28.69552017575814418, -279.3431013164529872, -236.8249705724439025 ) ) ;
#2656=CARTESIAN_POINT ( 'NONE',  ( 24.61681697343333042, -280.6728910039685729, -310.1601392661329442 ) ) ;
#2657=CARTESIAN_POINT ( 'NONE',  ( -35.88117069322078123, -284.1504598104225465, -195.9354432803787347 ) ) ;
#2658=CARTESIAN_POINT ( 'NONE',  ( -94.95184532012282830, -291.8888978003984676, -318.4024147159449285 ) ) ;
#2659=CARTESIAN_POINT ( 'NONE',  ( 18.25531823328056547, -282.0782529815833186, -222.4241710317243985 ) ) ;
#2660=CARTESIAN_POINT ( 'NONE',  ( -109.1155130956874899, -270.8344936138795447, -248.4232685986743832 ) ) ;
#2661=CARTESIAN_POINT ( 'NONE',  ( -35.93461544123370999, -281.4346933404005426, -346.5611091600961231 ) ) ;
#2662=CARTESIAN_POINT ( 'NONE',  ( 21.61570878164945952, -296.1889464444973328, -316.7393043373006094 ) ) ;
#2663=CARTESIAN_POINT ( 'NONE',  ( -33.93793638153591274, -278.3342854409783627, -194.4507207524731029 ) ) ;
#2664=CARTESIAN_POINT ( 'NONE',  ( -105.0392711043689786, -286.9816329592233046, -237.6951217885156780 ) ) ;
#2666=CARTESIAN_POINT ( 'NONE',  ( -55.85998831275767174, -293.7358328630814981, -197.0515634965084359 ) ) ;
#2667=CARTESIAN_POINT ( 'NONE',  ( 20.71399985140468303, -274.2066185410543540, -317.8633044961467249 ) ) ;
#2668=CARTESIAN_POINT ( 'NONE',  ( -85.07238799403340579, -288.8888079768875627, -330.6447916969686389 ) ) ;
#2669=CARTESIAN_POINT ( 'NONE',  ( 23.25634651762551997, -291.3710558232440349, -228.2161990809829035 ) ) ;
#2671=CARTESIAN_POINT ( 'NONE',  ( 16.88377877123530268, -274.9440314979038362, -319.9867466582619500 ) ) ;
#2672=CARTESIAN_POINT ( 'NONE',  ( -58.78733662842336116, -293.4720876267901417, -341.4311549408715223 ) ) ;
#2673=CARTESIAN_POINT ( 'NONE',  ( -100.7208091274395372, -291.3586604831730824, -307.6679269964687364 ) ) ;
#2676=CARTESIAN_POINT ( 'NONE',  ( 36.42133837648591310, -292.2788570749874566, -289.8988226797948187 ) ) ;
#2677=CARTESIAN_POINT ( 'NONE',  ( -19.64352469057129724, -287.8836886899214846, -198.7146595968324050 ) ) ;
#2678=CARTESIAN_POINT ( 'NONE',  ( -54.29759832383494711, -287.5067586405085649, -344.4858329171612468 ) ) ;
#2679=CARTESIAN_POINT ( 'NONE',  ( -11.83462947236000140, -287.8161317901507914, -201.3338460998832602 ) ) ;
#2680=CARTESIAN_POINT ( 'NONE',  ( 83.14890176555634582, -299.5541904835127980, -193.4651424135224147 ) ) ;
#2681=CARTESIAN_POINT ( 'NONE',  ( 25.84064955516008055, -288.8613487350610853, -307.3475045084510953 ) ) ;
#2682=CARTESIAN_POINT ( 'NONE',  ( -30.71004081858468382, -296.9485891865484177, -345.4239443177176554 ) ) ;
#2684=CARTESIAN_POINT ( 'NONE',  ( 19.97936702463683645, -288.0645513802183473, -219.4664596893020132 ) ) ;
#2685=CARTESIAN_POINT ( 'NONE',  ( -86.18337649788358590, -275.8028604735632143, -328.0820451556562602 ) ) ;
#2686=CARTESIAN_POINT ( 'NONE',  ( -96.13029495545859504, -278.2155036421382306, -320.0769888323100076 ) ) ;
#2687=CARTESIAN_POINT ( 'NONE',  ( 19.14753053243669711, -280.5063427849576669, -218.0666525879390747 ) ) ;
#2688=CARTESIAN_POINT ( 'NONE',  ( -111.3195000378592141, -274.5794567822068757, -262.0786474947299212 ) ) ;
#2689=CARTESIAN_POINT ( 'NONE',  ( -68.35200798006037815, -283.6446333426938509, -202.0723088026354617 ) ) ;
#2691=CARTESIAN_POINT ( 'NONE',  ( -60.08998674262525697, -277.8938816083247616, -199.6430583925055657 ) ) ;
#2692=CARTESIAN_POINT ( 'NONE',  ( -91.99211653074637240, -281.8321099976639061, -321.7446551986965915 ) ) ;
#2694=CARTESIAN_POINT ( 'NONE',  ( -59.48249724873398492, -275.8136620113664321, -343.3850377219923757 ) ) ;
#2695=CARTESIAN_POINT ( 'NONE',  ( -110.4902678018330562, -297.9500757429140663, -279.7128525874268803 ) ) ;
#2696=CARTESIAN_POINT ( 'NONE',  ( 36.17838733200018453, -280.7494716919017037, -292.3677470392498776 ) ) ;
#2697=CARTESIAN_POINT ( 'NONE',  ( -105.1753486792967323, -297.1248144635013659, -297.9655482751671229 ) ) ;
#2698=CARTESIAN_POINT ( 'NONE',  ( -46.09021219033369476, -299.2585613696900282, -194.3561062476720451 ) ) ;
#2699=CARTESIAN_POINT ( 'NONE',  ( -81.08027928402636064, -273.1063478667110758, -211.8252506950797169 ) ) ;
#2700=CARTESIAN_POINT ( 'NONE',  ( 0.9077138322254096892, -294.5626779567892299, -205.8476854246210337 ) ) ;
#2701=CARTESIAN_POINT ( 'NONE',  ( 2.739199855610745971, -286.7409349505085174, -204.6152324763273782 ) ) ;
#2702=CARTESIAN_POINT ( 'NONE',  ( -95.68955208083121988, -277.2894252167806712, -222.3322314468233856 ) ) ;
#2703=CARTESIAN_POINT ( 'NONE',  ( -82.85435356233550408, -289.4890413853051996, -332.4706855374815291 ) ) ;
#2704=CARTESIAN_POINT ( 'NONE',  ( -21.08874187012393620, -287.8971944043843223, -341.7701495908441416 ) ) ;
#2705=CARTESIAN_POINT ( 'NONE',  ( 7.671467575295017660, -290.6659425368728762, -210.3061573505725050 ) ) ;
#2707=CARTESIAN_POINT ( 'NONE',  ( 207.9737475149031525, 296.4638663539913637, -68.98948423471202318 ) ) ;
#2708=CARTESIAN_POINT ( 'NONE',  ( -37.27425110047372669, -288.5589369964210960, -343.4226255807204211 ) ) ;
#2710=CARTESIAN_POINT ( 'NONE',  ( -96.98198631410483017, -284.8429599868558171, -318.7124702920821733 ) ) ;
#2711=CARTESIAN_POINT ( 'NONE',  ( -19.43000539545679572, -291.3357273645840451, -195.6606881735908132 ) ) ;
#2713=CARTESIAN_POINT ( 'NONE',  ( -41.52531235935615683, -284.4188357550344790, -346.8054895221640663 ) ) ;
#2715=CARTESIAN_POINT ( 'NONE',  ( -4.829069549432396968, -282.4448676174676507, -335.7211123016501801 ) ) ;
#2716=CARTESIAN_POINT ( 'NONE',  ( -111.6220714087064039, -296.8084282231895372, -249.8804470308761552 ) ) ;
#2717=CARTESIAN_POINT ( 'NONE',  ( 35.19664998397951194, -277.0260885663154795, -282.4771392354473392 ) ) ;
#2718=CARTESIAN_POINT ( 'NONE',  ( -9.081911065104558034, -290.4434890716537438, -201.2175371920630766 ) ) ;
#2719=CARTESIAN_POINT ( 'NONE',  ( -62.14954914469169722, -272.5171341220921590, -201.2836170738869157 ) ) ;
#2722=CARTESIAN_POINT ( 'NONE',  ( -88.70544114177731387, -287.2445392621377209, -216.4808775858933529 ) ) ;
#2723=CARTESIAN_POINT ( 'NONE',  ( -47.57665820279462565, -296.2590341920533774, -346.3659740272857448 ) ) ;
#2724=CARTESIAN_POINT ( 'NONE',  ( -103.1007377632841582, -284.7704860687312589, -302.4091723047908431 ) ) ;
#2725=CARTESIAN_POINT ( 'NONE',  ( -28.63965096828158963, -276.0032425536001597, -346.6844086941429737 ) ) ;
#2726=CARTESIAN_POINT ( 'NONE',  ( 29.38307255683859154, -293.7062620986482671, -232.1365513208092182 ) ) ;
#2727=CARTESIAN_POINT ( 'NONE',  ( 22.89406244231098597, -285.0688448791775045, -224.3837900243584045 ) ) ;
#2728=CARTESIAN_POINT ( 'NONE',  ( 36.35068573455915697, -294.1668587906486891, -292.7942859032173146 ) ) ;
#2729=CARTESIAN_POINT ( 'NONE',  ( -108.6824671081372031, -290.6793230287998426, -285.9942879991552331 ) ) ;
#2732=CARTESIAN_POINT ( 'NONE',  ( -62.37129463845912625, -182.9780070361101991, -358.6976082868463891 ) ) ;
#2733=CARTESIAN_POINT ( 'NONE',  ( -110.0192286520845073, -285.7767764354590554, -293.6567987104924669 ) ) ;
#2734=CARTESIAN_POINT ( 'NONE',  ( 36.60358173371529489, -278.6237833571632905, -234.7871824221999191 ) ) ;
#2736=CARTESIAN_POINT ( 'NONE',  ( -80.82047541408202562, -282.5779316952025511, -329.4481958337401011 ) ) ;
#2737=CARTESIAN_POINT ( 'NONE',  ( -91.31723784293288304, -277.4609677338074221, -325.3209727301505154 ) ) ;
#2738=CARTESIAN_POINT ( 'NONE',  ( 35.54026667780902216, -283.3338264541879425, -253.3832693056166079 ) ) ;
#2739=CARTESIAN_POINT ( 'NONE',  ( -81.56226884185248593, -220.3210169592839520, -351.0985766935151560 ) ) ;
#2740=CARTESIAN_POINT ( 'NONE',  ( 4.209938585483945062, -281.0789763095443732, -334.5490505033449722 ) ) ;
#2741=CARTESIAN_POINT ( 'NONE',  ( 7.944381906164617924, -284.6940646746120933, -210.9576313398227398 ) ) ;
#2742=CARTESIAN_POINT ( 'NONE',  ( -87.24096160769006758, -275.2262057935647590, -213.2793377503666079 ) ) ;
#2743=CARTESIAN_POINT ( 'NONE',  ( -7.957809596465249768, -295.1488612952133508, -337.2669747142366532 ) ) ;
#2744=CARTESIAN_POINT ( 'NONE',  ( 23.00236286806038422, -291.6559641898066957, -228.3885197761897246 ) ) ;
#2745=CARTESIAN_POINT ( 'NONE',  ( -84.79694765792467592, -278.3380713043167702, -330.9375515814594451 ) ) ;
#2746=CARTESIAN_POINT ( 'NONE',  ( 32.89785625263545654, -275.8155770141138419, -290.2916489331177559 ) ) ;
#2747=CARTESIAN_POINT ( 'NONE',  ( 33.43361238478622965, -274.0938120734829226, -240.6883679346808265 ) ) ;
#2749=CARTESIAN_POINT ( 'NONE',  ( 29.52501195980105564, -274.0023074647206158, -304.4424623720775571 ) ) ;
#2750=CARTESIAN_POINT ( 'NONE',  ( -13.94507580407868197, -296.1796593822725185, -343.1017824146418320 ) ) ;
#2753=CARTESIAN_POINT ( 'NONE',  ( -106.4605913472635450, -285.3062854420732037, -294.9417921748872118 ) ) ;
#2754=CARTESIAN_POINT ( 'NONE',  ( -113.3406613365604159, -286.2808928153247621, -272.8388528738504419 ) ) ;
#2755=CARTESIAN_POINT ( 'NONE',  ( -72.41564051331070573, -284.9235527089034576, -206.2086614824857804 ) ) ;
#2756=CARTESIAN_POINT ( 'NONE',  ( 32.00658406916826948, -274.2864893383505773, -295.7534321924774758 ) ) ;
#2757=CARTESIAN_POINT ( 'NONE',  ( 35.92642766521837672, -283.5675041894049855, -282.3046070428194980 ) ) ;
#2758=CARTESIAN_POINT ( 'NONE',  ( -18.86159556224215450, -275.2897404266887520, -341.6997014127180705 ) ) ;
#2759=CARTESIAN_POINT ( 'NONE',  ( -56.66848074325722706, -278.3867687708254266, -341.1294742975649683 ) ) ;
#2761=CARTESIAN_POINT ( 'NONE',  ( -82.15299265512079785, -280.2607854637705600, -207.9423156702887354 ) ) ;
#2762=CARTESIAN_POINT ( 'NONE',  ( -59.29058944443922741, -280.2677606479604719, -196.6198597829484811 ) ) ;
#2765=CARTESIAN_POINT ( 'NONE',  ( 36.90269544335986041, -289.6045155762329841, -285.4632770918300366 ) ) ;
#2766=CARTESIAN_POINT ( 'NONE',  ( -109.5238969235007715, -295.5922831480214086, -282.2914236355272237 ) ) ;
#2767=CARTESIAN_POINT ( 'NONE',  ( -82.79907439499299926, -289.0043862434667403, -332.3848224111608829 ) ) ;
#2768=CARTESIAN_POINT ( 'NONE',  ( 16.41722005353504699, -285.4095778059436839, -220.0896226530646231 ) ) ;
#2769=CARTESIAN_POINT ( 'NONE',  ( -111.1348562872789358, -288.7095986691595044, -276.6946171438947886 ) ) ;
#2771=CARTESIAN_POINT ( 'NONE',  ( 13.40305642130455155, -287.9862516103727330, -217.2617747311107337 ) ) ;
#2772=CARTESIAN_POINT ( 'NONE',  ( -64.39798358256457789, -275.4049527941206748, -340.3656341580193612 ) ) ;
#2773=CARTESIAN_POINT ( 'NONE',  ( -17.94780361404993840, -287.2060191304763066, -344.0518039034200797 ) ) ;
#2774=CARTESIAN_POINT ( 'NONE',  ( -13.36776127044652007, -288.3636626835776156, -199.2960006397966310 ) ) ;
#2775=CARTESIAN_POINT ( 'NONE',  ( -69.86933689767057842, -287.4792636309319960, -338.1394199468418265 ) ) ;
#2776=CARTESIAN_POINT ( 'NONE',  ( -56.36851980457477396, -284.2446842523890496, -341.0816141660307608 ) ) ;
#2777=CARTESIAN_POINT ( 'NONE',  ( -105.6063829402270642, -292.9660349814196820, -238.7733616052207140 ) ) ;
#2778=CARTESIAN_POINT ( 'NONE',  ( 82.16487609371904455, -298.2963867135958935, -193.7956126067913658 ) ) ;
#2780=CARTESIAN_POINT ( 'NONE',  ( -75.08227273479333519, -299.4740249117562598, -204.8414279612577786 ) ) ;
#2781=CARTESIAN_POINT ( 'NONE',  ( -36.99732744133339679, -279.2537393160829993, -197.2004513985829135 ) ) ;
#2782=CARTESIAN_POINT ( 'NONE',  ( 31.87685371402460532, -279.1749930218220470, -241.4856534825018741 ) ) ;
#2783=CARTESIAN_POINT ( 'NONE',  ( 38.65532623992585570, -292.8914511685017033, -281.7017883206525539 ) ) ;
#2784=CARTESIAN_POINT ( 'NONE',  ( -97.08625777033148552, -271.3964263819379426, -226.5889108564023218 ) ) ;
#2785=CARTESIAN_POINT ( 'NONE',  ( 21.13884602993729445, -274.2693853264119070, -316.4396442319369385 ) ) ;
#2786=CARTESIAN_POINT ( 'NONE',  ( -97.57803656960989258, -297.2841462128938588, -312.4660731617087208 ) ) ;
#2788=CARTESIAN_POINT ( 'NONE',  ( -9.406579345672197334, -296.8757723994409616, -194.0615142604495134 ) ) ;
#2789=CARTESIAN_POINT ( 'NONE',  ( 36.79030919207632166, -292.0042241912066743, -287.1056707402462962 ) ) ;
#2790=CARTESIAN_POINT ( 'NONE',  ( -52.50879800661054730, -293.2794828443963411, -198.2995316729631838 ) ) ;
#2792=CARTESIAN_POINT ( 'NONE',  ( 28.54441147741274065, -294.7858595178612973, -302.2839908343195248 ) ) ;
#2794=CARTESIAN_POINT ( 'NONE',  ( -69.78531745579915935, -281.4972470165252503, -338.3886424621617834 ) ) ;
#2795=CARTESIAN_POINT ( 'NONE',  ( 8.228166959662209123, -294.4088991144729448, -327.4557880836728145 ) ) ;
#2796=CARTESIAN_POINT ( 'NONE',  ( 11.49260014145638031, -282.3965537359416658, -329.9633923317568360 ) ) ;
#2797=CARTESIAN_POINT ( 'NONE',  ( 36.26899276346060219, -283.2543199970677961, -253.2520769356646042 ) ) ;
#2798=CARTESIAN_POINT ( 'NONE',  ( -85.49637932775860349, -285.0734653645772596, -210.3038855903564013 ) ) ;
#2799=CARTESIAN_POINT ( 'NONE',  ( -111.9526576019002704, -288.4696180730693413, -276.7619910168854744 ) ) ;
#2800=CARTESIAN_POINT ( 'NONE',  ( 38.18225885682601728, -280.1696088025414042, -281.2624652323590908 ) ) ;
#2801=CARTESIAN_POINT ( 'NONE',  ( 23.95457119407326019, -285.6771258154308271, -229.7225497859528787 ) ) ;
#2802=CARTESIAN_POINT ( 'NONE',  ( 12.20560971778196091, -287.3014911065483830, -328.8979149220623412 ) ) ;
#2804=CARTESIAN_POINT ( 'NONE',  ( -45.15539717101938777, -296.7527448739286910, -343.7973404873493450 ) ) ;
#2805=CARTESIAN_POINT ( 'NONE',  ( -79.88295558156283960, -279.0401950349207709, -333.8980084025261021 ) ) ;
#2806=CARTESIAN_POINT ( 'NONE',  ( 36.45459683255092642, -291.7671284948152675, -285.6095067920849715 ) ) ;
#2807=CARTESIAN_POINT ( 'NONE',  ( -74.51289745166468492, -279.2100307053224242, -207.4508765930658285 ) ) ;
#2809=CARTESIAN_POINT ( 'NONE',  ( 4.139746364101549503, -292.7609560338043480, -205.4265875402523989 ) ) ;
#2810=CARTESIAN_POINT ( 'NONE',  ( -62.69480716997583158, -283.8045586427365947, -199.1815270844266763 ) ) ;
#2811=CARTESIAN_POINT ( 'NONE',  ( -50.92474409682142777, -279.2258922889168957, -344.1208736928884377 ) ) ;
#2813=CARTESIAN_POINT ( 'NONE',  ( -47.83857301979428200, -294.2475225237496375, -342.8916930074684615 ) ) ;
#2814=CARTESIAN_POINT ( 'NONE',  ( -54.12226128174090434, -295.8364965076098656, -197.2624626393473477 ) ) ;
#2817=CARTESIAN_POINT ( 'NONE',  ( 37.15999247101181169, -283.4724467757494040, -265.7410963307617067 ) ) ;
#2818=CARTESIAN_POINT ( 'NONE',  ( -94.82573711846927722, -295.4244564360678282, -315.4562832795411964 ) ) ;
#2820=CARTESIAN_POINT ( 'NONE',  ( -54.49178911615187104, -274.7666405000204577, -345.3538533559490702 ) ) ;
#2821=CARTESIAN_POINT ( 'NONE',  ( -36.17674695991064482, -297.1251560531955533, -193.5965911883371859 ) ) ;
#2822=CARTESIAN_POINT ( 'NONE',  ( -9.725616075764879298, -290.0139872273785500, -341.7099103643789704 ) ) ;
#2823=CARTESIAN_POINT ( 'NONE',  ( -50.75354785169238170, -289.0614556014573964, -342.1701823921899290 ) ) ;
#2824=CARTESIAN_POINT ( 'NONE',  ( -93.63221653140652734, -280.7419848737471852, -222.7803136771873085 ) ) ;
#2825=CARTESIAN_POINT ( 'NONE',  ( -109.3196191172755221, -274.3649467318228972, -254.0632777641390021 ) ) ;
#2826=CARTESIAN_POINT ( 'NONE',  ( -7.825759062145887235, -279.2426718483865784, -203.1466276485403739 ) ) ;
#2828=CARTESIAN_POINT ( 'NONE',  ( -70.71603551743220351, -297.2906472624725325, -200.9932721964837867 ) ) ;
#2829=CARTESIAN_POINT ( 'NONE',  ( -49.95634484765677286, -293.8102664243620552, -196.9454017739848837 ) ) ;
#2831=ADVANCED_FACE ( 'NONE', ( #87479 ), #44889, .F. ) ;
#2832=CARTESIAN_POINT ( 'NONE',  ( -104.8003338258955068, -291.5824069597491075, -242.0650969702264774 ) ) ;
#2834=CARTESIAN_POINT ( 'NONE',  ( -8.951720534258400974, -290.5591488951637302, -200.1164417439935903 ) ) ;
#2836=CARTESIAN_POINT ( 'NONE',  ( -49.95340010446486190, -297.5534975373815882, -198.4373214309470370 ) ) ;
#2839=CARTESIAN_POINT ( 'NONE',  ( -96.05788420657935944, -292.7337038235289697, -221.6057418116824920 ) ) ;
#2840=CARTESIAN_POINT ( 'NONE',  ( -119.3990491898856732, -287.0519495502701943, -270.3937649182068412 ) ) ;
#2841=CARTESIAN_POINT ( 'NONE',  ( 1.088840022142868680, -288.5661438620001036, -206.0891764034962819 ) ) ;
#2842=CARTESIAN_POINT ( 'NONE',  ( -9.325044589421599639, -274.6849535557645936, -339.7659108541024011 ) ) ;
#2843=CARTESIAN_POINT ( 'NONE',  ( 34.23804555264609206, -277.2051688667561962, -249.7405601132960840 ) ) ;
#2844=CARTESIAN_POINT ( 'NONE',  ( -70.84739378904981777, -289.6864163923318074, -203.8879452476151926 ) ) ;
#2845=CARTESIAN_POINT ( 'NONE',  ( -100.8686835716760726, -280.9646906277680500, -228.9790026064348467 ) ) ;
#2848=CARTESIAN_POINT ( 'NONE',  ( -64.10039669164578413, -282.7592697003752846, -338.3895298887953231 ) ) ;
#2849=CARTESIAN_POINT ( 'NONE',  ( -93.09976414047308424, -278.9092381510017162, -323.0921328405184454 ) ) ;
#2850=CARTESIAN_POINT ( 'NONE',  ( 1.187602918908520655, -279.3492116665115077, -204.0927027560734643 ) ) ;
#2851=CARTESIAN_POINT ( 'NONE',  ( -71.49185695405026308, -195.2781849387351940, -357.0959408212342510 ) ) ;
#2852=CARTESIAN_POINT ( 'NONE',  ( 27.45667162853909105, -277.0355815205247723, -311.6180747683662275 ) ) ;
#2853=CARTESIAN_POINT ( 'NONE',  ( -67.28160103364130862, -275.1867171468312563, -200.1734403777877844 ) ) ;
#2854=CARTESIAN_POINT ( 'NONE',  ( -92.08974858914540107, -275.6948066931273047, -226.7417163044926838 ) ) ;
#2856=CARTESIAN_POINT ( 'NONE',  ( -78.33593093052400036, -290.6974386804960204, -331.1980336568678922 ) ) ;
#2857=CARTESIAN_POINT ( 'NONE',  ( -45.88922343606126475, -290.9191123339097089, -345.9179412343022477 ) ) ;
#2858=CARTESIAN_POINT ( 'NONE',  ( -65.35836473592824802, -291.0245960728885848, -202.8275208056123233 ) ) ;
#2859=CARTESIAN_POINT ( 'NONE',  ( 2.714328192050878830, -286.0820139869255740, -204.6721425118038837 ) ) ;
#2860=CARTESIAN_POINT ( 'NONE',  ( -29.37836264791282304, -281.3496091152964027, -343.7812803602099621 ) ) ;
#2861=CARTESIAN_POINT ( 'NONE',  ( -5.237154793796259256, -290.4854685085708752, -337.2951426109901263 ) ) ;
#2862=CARTESIAN_POINT ( 'NONE',  ( -91.26183937304736560, -282.3164937269717711, -320.5938397536647244 ) ) ;
#2863=CARTESIAN_POINT ( 'NONE',  ( 15.60310234595508128, -282.1355650153560646, -219.3169602091612376 ) ) ;
#2864=CARTESIAN_POINT ( 'NONE',  ( 36.56115665267015657, -288.7549626652714778, -291.1744180273909137 ) ) ;
#2865=CARTESIAN_POINT ( 'NONE',  ( -103.4281870388300462, -279.4665099721584625, -239.0882953529059591 ) ) ;
#2866=CARTESIAN_POINT ( 'NONE',  ( 8.624982094127268795, -291.4608993500235670, -209.0162564729106123 ) ) ;
#2867=CARTESIAN_POINT ( 'NONE',  ( 37.21765845827852814, -288.1220925132266188, -251.7853039135123367 ) ) ;
#2868=CARTESIAN_POINT ( 'NONE',  ( 1.485204760623171083, -287.0488303815515678, -203.9229172603655513 ) ) ;
#2869=CARTESIAN_POINT ( 'NONE',  ( -61.53272083558573513, -283.5419036321370072, -339.2895632518391835 ) ) ;
#2872=CARTESIAN_POINT ( 'NONE',  ( -5.150820151708191297, -294.3317621872541281, -201.7750207701828344 ) ) ;
#2873=CARTESIAN_POINT ( 'NONE',  ( 38.74476234958408583, -292.3439164272979269, -278.8568525136179801 ) ) ;
#2874=CARTESIAN_POINT ( 'NONE',  ( 15.76026168670163408, -275.3356033178822599, -320.7951352683645041 ) ) ;
#2875=CARTESIAN_POINT ( 'NONE',  ( -95.48856867577825369, -296.5821054423128658, -219.9601463135191750 ) ) ;
#2876=CARTESIAN_POINT ( 'NONE',  ( 11.40379034033410299, -291.2220414918509164, -215.0247091504053571 ) ) ;
#2877=CARTESIAN_POINT ( 'NONE',  ( -107.6626292927897737, -295.0961193701960497, -247.1132791505773412 ) ) ;
#2878=CARTESIAN_POINT ( 'NONE',  ( -62.95358841780969783, -292.9161529783538640, -201.5776775115582211 ) ) ;
#2879=CARTESIAN_POINT ( 'NONE',  ( -4.707777516483687918, -293.5720805570799143, -204.7022333330794197 ) ) ;
#2881=CARTESIAN_POINT ( 'NONE',  ( -11.70697373698338950, -292.7191181847800863, -341.0767123416845266 ) ) ;
#2882=CARTESIAN_POINT ( 'NONE',  ( -93.46545006823660628, -299.2444835154307725, -220.5913497278921795 ) ) ;
#2883=CARTESIAN_POINT ( 'NONE',  ( 32.49436237846204989, -288.2015092053195531, -248.2662015151656192 ) ) ;
#2884=CARTESIAN_POINT ( 'NONE',  ( -20.46931860436149009, -278.8165469422323213, -343.8566872408301265 ) ) ;
#2885=CARTESIAN_POINT ( 'NONE',  ( -41.37894363133016640, -275.8968223335654670, -346.8707251310198103 ) ) ;
#2886=CARTESIAN_POINT ( 'NONE',  ( -94.06446177829603528, -272.6080721097270043, -218.4201888353314018 ) ) ;
#2887=CARTESIAN_POINT ( 'NONE',  ( -2.977954173149480077, -280.6743074147379957, -336.4090794574188976 ) ) ;
#2888=CARTESIAN_POINT ( 'NONE',  ( -95.55139297034149592, -276.2824067017272682, -319.5551605005184683 ) ) ;
#2890=CARTESIAN_POINT ( 'NONE',  ( -101.6379645964201188, -295.7202586623055822, -234.7628897645957409 ) ) ;
#2892=CARTESIAN_POINT ( 'NONE',  ( 51.90681045958935158, -300.0003654427256947, -197.1871290551031848 ) ) ;
#2894=CARTESIAN_POINT ( 'NONE',  ( -83.24402990789482715, -289.4474636461882824, -210.5343208057203697 ) ) ;
#2895=CARTESIAN_POINT ( 'NONE',  ( -62.02769912935531949, -273.5553623970110948, -201.6617623974533160 ) ) ;
#2896=CARTESIAN_POINT ( 'NONE',  ( -3.060732189554848492, -288.6118421495224311, -339.3236633873809751 ) ) ;
#2897=CARTESIAN_POINT ( 'NONE',  ( -94.64693616848038005, -275.2241708497983836, -221.6983236229328043 ) ) ;
#2898=CARTESIAN_POINT ( 'NONE',  ( -93.19672922290135375, -295.2467577503680900, -220.5590682967963403 ) ) ;
#2899=CARTESIAN_POINT ( 'NONE',  ( -81.47718342649301349, -282.8326430093590602, -333.3243269062834884 ) ) ;
#2901=CARTESIAN_POINT ( 'NONE',  ( 34.73986262293673377, -279.2832123456855697, -249.4613584316390700 ) ) ;
#2903=CARTESIAN_POINT ( 'NONE',  ( -70.38581510824025145, -290.4013790358661140, -204.8232131397174385 ) ) ;
#2904=CARTESIAN_POINT ( 'NONE',  ( -109.2962303322233026, -282.4547446666628616, -288.6206652414547875 ) ) ;
#2906=CARTESIAN_POINT ( 'NONE',  ( -71.09870476466221589, -289.6064229077545065, -203.3875016063779526 ) ) ;
#2907=CARTESIAN_POINT ( 'NONE',  ( -87.82220854867985338, -274.8516771856002379, -216.6030027083346852 ) ) ;
#2908=CARTESIAN_POINT ( 'NONE',  ( 11.25262060570510947, -283.6014355524578150, -329.6463279634551782 ) ) ;
#2909=CARTESIAN_POINT ( 'NONE',  ( -82.69584842527063984, -271.5179643175806063, -209.8612594424555198 ) ) ;
#2910=CARTESIAN_POINT ( 'NONE',  ( -64.05537194972967541, -283.4105777766824303, -338.2977041332143244 ) ) ;
#2911=CARTESIAN_POINT ( 'NONE',  ( 12.15735637397209068, -277.7729995579064735, -324.8840983225068726 ) ) ;
#2912=CARTESIAN_POINT ( 'NONE',  ( -39.15153233043744052, -277.8782774392157648, -343.5002062653364305 ) ) ;
#2913=CARTESIAN_POINT ( 'NONE',  ( -3.764762803192364782, -284.6093846415869280, -337.4394659220541257 ) ) ;
#2914=EDGE_CURVE ( 'NONE', #37641, #1315, #66663, .T. ) ;
#2917=CARTESIAN_POINT ( 'NONE',  ( -22.09962252229478707, -294.6953883675424777, -345.8374657661136098 ) ) ;
#2918=CARTESIAN_POINT ( 'NONE',  ( 17.15852877712842073, -288.8141928387911435, -219.3366568809630053 ) ) ;
#2920=CARTESIAN_POINT ( 'NONE',  ( 44.71564893372296723, -285.0523547857347353, -270.3937649182068412 ) ) ;
#2921=CARTESIAN_POINT ( 'NONE',  ( -64.61947273876879194, -278.6246938338379096, -198.6293515077563256 ) ) ;
#2922=CARTESIAN_POINT ( 'NONE',  ( -108.7172567006733743, -289.2947493576018019, -243.5280846392117269 ) ) ;
#2923=CARTESIAN_POINT ( 'NONE',  ( -95.51620273670941685, -286.7038534672208812, -225.1030815780964360 ) ) ;
#2924=CARTESIAN_POINT ( 'NONE',  ( -106.2025032871872980, -279.9544073437096472, -297.4934566202261408 ) ) ;
#2925=CARTESIAN_POINT ( 'NONE',  ( -106.1563940164742803, -286.4068372814649592, -237.1475033595592095 ) ) ;
#2926=CARTESIAN_POINT ( 'NONE',  ( -15.52709920383375142, -284.7699772989835765, -342.1185136498224324 ) ) ;
#2927=CARTESIAN_POINT ( 'NONE',  ( -31.44814834119044633, -277.1464904308163000, -347.1878648014589999 ) ) ;
#2928=CARTESIAN_POINT ( 'NONE',  ( -89.21368040031019575, -277.5917971751738946, -327.2671604308478095 ) ) ;
#2929=CARTESIAN_POINT ( 'NONE',  ( -96.44706004355793993, -299.0968105714748049, -225.0869355814819528 ) ) ;
#2932=CARTESIAN_POINT ( 'NONE',  ( -106.6379572354042296, -280.6233781216988064, -303.7686719486574702 ) ) ;
#2933=CARTESIAN_POINT ( 'NONE',  ( 29.45481597813228802, -297.0194551764546418, -194.6172037023857513 ) ) ;
#2935=CARTESIAN_POINT ( 'NONE',  ( -37.81644747580428145, -276.5658722141536714, -343.4335775399458157 ) ) ;
#2936=CARTESIAN_POINT ( 'NONE',  ( 24.15190359836281786, -276.1466954785532266, -224.6823984261923499 ) ) ;
#2937=CARTESIAN_POINT ( 'NONE',  ( 35.38230468208542590, -280.9232887556263449, -295.1034455707778079 ) ) ;
#2938=CARTESIAN_POINT ( 'NONE',  ( 14.81312134196681640, -290.0649169452819365, -322.8763406324623020 ) ) ;
#2939=CARTESIAN_POINT ( 'NONE',  ( -95.96620879823493055, -297.4090596858279127, -319.2268452488467005 ) ) ;
#2940=CARTESIAN_POINT ( 'NONE',  ( -113.5466448117420839, -297.6591900471490817, -278.1595231856105102 ) ) ;
#2941=CARTESIAN_POINT ( 'NONE',  ( -11.65423065400196023, -294.3874482102523871, -200.0194642710369521 ) ) ;
#2942=CARTESIAN_POINT ( 'NONE',  ( 30.64877523258950376, -279.1391369767742390, -238.9746644816205219 ) ) ;
#2943=CARTESIAN_POINT ( 'NONE',  ( 29.05495563625945366, -283.0228044141385908, -236.5898266888796684 ) ) ;
#2944=CARTESIAN_POINT ( 'NONE',  ( -44.68731909621574516, -296.0384519634630465, -196.2330519449467374 ) ) ;
#2945=CARTESIAN_POINT ( 'NONE',  ( -111.5849307654610385, -286.3691074003725134, -253.2035213163013054 ) ) ;
#2946=CARTESIAN_POINT ( 'NONE',  ( -2.025449827848527118, -285.4514203212203256, -206.0625150002080659 ) ) ;
#2947=CARTESIAN_POINT ( 'NONE',  ( 21.89749367432979454, -280.2407708675747813, -221.3302021775997162 ) ) ;
#2948=CARTESIAN_POINT ( 'NONE',  ( -93.70700619081699756, -240.9337940567206431, -341.5190362321769157 ) ) ;
#2950=CARTESIAN_POINT ( 'NONE',  ( -69.12886551661786427, -288.0368317553940187, -339.8605567356493111 ) ) ;
#2951=CARTESIAN_POINT ( 'NONE',  ( 24.97097506146832657, -286.6945253799232773, -232.2925220345383082 ) ) ;
#2952=ORIENTED_EDGE ( 'NONE', *, *, #80976, .T. ) ;
#2953=CARTESIAN_POINT ( 'NONE',  ( -113.2912712511572408, -285.4935443032257467, -281.3731746439570429 ) ) ;
#2954=CARTESIAN_POINT ( 'NONE',  ( 33.26372301889318805, -276.1313242869352962, -288.9880261822770535 ) ) ;
#2956=CARTESIAN_POINT ( 'NONE',  ( -19.44550728358895242, -291.1973302276585400, -195.7329335394500447 ) ) ;
#2957=CARTESIAN_POINT ( 'NONE',  ( 28.22244103946771432, -282.7304047362337656, -310.6448302517616753 ) ) ;
#2958=CARTESIAN_POINT ( 'NONE',  ( -101.3205667520087445, -280.6244515284915906, -228.6792664564569861 ) ) ;
#2959=CARTESIAN_POINT ( 'NONE',  ( 21.95170591714795805, -281.2253059536230353, -221.2689975232774486 ) ) ;
#2960=CARTESIAN_POINT ( 'NONE',  ( 30.91033621190086578, -290.8380690714489560, -254.8156830097664738 ) ) ;
#2961=CARTESIAN_POINT ( 'NONE',  ( 6.325340719953564061, -58.69197721219502029, -354.8253570307668952 ) ) ;
#2963=CARTESIAN_POINT ( 'NONE',  ( 16.94494931043544028, -278.2765412746037441, -321.8682836903628299 ) ) ;
#2964=CARTESIAN_POINT ( 'NONE',  ( 201.1675596189675446, 293.6556537245446634, -83.10562796347613812 ) ) ;
#2966=CARTESIAN_POINT ( 'NONE',  ( 25.50188153274858394, -280.1183605235837035, -310.7367447317829487 ) ) ;
#2967=CARTESIAN_POINT ( 'NONE',  ( -101.2997446411217908, -296.3839126046775050, -234.9596884921501214 ) ) ;
#2968=CARTESIAN_POINT ( 'NONE',  ( 38.26592855160097884, -292.8814704008326544, -256.1128412858878960 ) ) ;
#2970=CARTESIAN_POINT ( 'NONE',  ( -67.92481853885293219, -296.2333603907616748, -200.2813436115579009 ) ) ;
#2971=CARTESIAN_POINT ( 'NONE',  ( -73.95941970419592337, -287.9470323679709054, -334.4505129913720225 ) ) ;
#2972=CARTESIAN_POINT ( 'NONE',  ( -25.99563728367191828, -296.7665640718874442, -343.7241354788083640 ) ) ;
#2973=CARTESIAN_POINT ( 'NONE',  ( -41.36657001774556619, -287.3156292685786184, -196.9656769640162395 ) ) ;
#2975=CARTESIAN_POINT ( 'NONE',  ( -3.436110940620233478, -293.4300646426044636, -201.4755056033205278 ) ) ;
#2976=CARTESIAN_POINT ( 'NONE',  ( -106.2296571493007349, -284.7190558751621552, -294.8517802936671615 ) ) ;
#2977=CARTESIAN_POINT ( 'NONE',  ( -97.02726496196710571, -295.9939609678064016, -222.3440161226215253 ) ) ;
#2978=CARTESIAN_POINT ( 'NONE',  ( -77.09449430967256944, -292.3369076640341859, -204.5435781759580607 ) ) ;
#2979=CARTESIAN_POINT ( 'NONE',  ( -5.917812314285831654, -292.9465971988785213, -200.1181710203466366 ) ) ;
#2980=CARTESIAN_POINT ( 'NONE',  ( -34.57587542716795781, -289.1832534903532519, -343.3582849914051849 ) ) ;
#2983=CARTESIAN_POINT ( 'NONE',  ( -70.21488714162688893, -299.4839891301380135, -202.0994225688680785 ) ) ;
#2984=CARTESIAN_POINT ( 'NONE',  ( -57.99970379579195878, -272.5861082653977405, -196.5411150402163685 ) ) ;
#2985=CARTESIAN_POINT ( 'NONE',  ( 5.720802865667158343, -281.5109840627208655, -329.5981780326182502 ) ) ;
#2987=CARTESIAN_POINT ( 'NONE',  ( 12.65986701365186384, -275.8839807285244206, -328.8364990110983399 ) ) ;
#2988=CARTESIAN_POINT ( 'NONE',  ( -106.1548794823400925, -271.3061729983235750, -243.5521685186124330 ) ) ;
#2989=CARTESIAN_POINT ( 'NONE',  ( -67.83496793265835834, -281.5080505367585033, -202.6640011536138957 ) ) ;
#2990=CARTESIAN_POINT ( 'NONE',  ( 33.69153331797667761, -273.9730815556033008, -291.9723621250579413 ) ) ;
#2991=CARTESIAN_POINT ( 'NONE',  ( -41.90829471547915830, -299.1984041650800350, -197.1062429286031090 ) ) ;
#2992=CARTESIAN_POINT ( 'NONE',  ( -98.04492213693521308, -274.0620976265568061, -229.3007920494205791 ) ) ;
#2993=CARTESIAN_POINT ( 'NONE',  ( -112.8122911223118194, -298.2863968740475684, -259.7484565993211731 ) ) ;
#2994=CARTESIAN_POINT ( 'NONE',  ( 1.590278049532844351, -272.5900234431163653, -205.8420674816332507 ) ) ;
#2995=CARTESIAN_POINT ( 'NONE',  ( 20.60907936929845974, -294.8300248985997314, -314.9416857134140741 ) ) ;
#2996=CARTESIAN_POINT ( 'NONE',  ( -17.25446246306490750, -290.8911275413054227, -199.5134797963687276 ) ) ;
#2998=CARTESIAN_POINT ( 'NONE',  ( 9.467932666813636544, -275.1689144392015578, -209.3006137211017688 ) ) ;
#2999=CARTESIAN_POINT ( 'NONE',  ( -62.03169170696425994, -273.8886687302750147, -201.6631971964509376 ) ) ;
#3000=CARTESIAN_POINT ( 'NONE',  ( -38.74043224664081464, -281.7541842362255124, -346.8551819548016510 ) ) ;
#3001=CARTESIAN_POINT ( 'NONE',  ( -22.43559455235949684, -296.8618801444668520, -344.0349697897236183 ) ) ;
#3003=CARTESIAN_POINT ( 'NONE',  ( -109.7706457989530122, -283.8852471624824148, -260.0339907911579189 ) ) ;
#3004=CARTESIAN_POINT ( 'NONE',  ( -106.5493604861856340, -282.1680181430447192, -299.8257300144005058 ) ) ;
#3005=ADVANCED_FACE ( 'NONE', ( #44406 ), #23254, .F. ) ;
#3006=CARTESIAN_POINT ( 'NONE',  ( 36.23238107834401944, -274.1073329748978153, -268.8679702717868736 ) ) ;
#3007=CARTESIAN_POINT ( 'NONE',  ( 10.88161637998043396, -282.7188842188192552, -212.8526851851519268 ) ) ;
#3010=CARTESIAN_POINT ( 'NONE',  ( -27.08382758656488676, -272.5802125551643371, -194.8018419186716415 ) ) ;
#3011=CARTESIAN_POINT ( 'NONE',  ( -64.41049912907440955, -279.4046283878169561, -340.5395785599721421 ) ) ;
#3013=CARTESIAN_POINT ( 'NONE',  ( -106.8919198422468355, -286.0877017183601652, -300.0258869104520727 ) ) ;
#3015=CARTESIAN_POINT ( 'NONE',  ( -112.3869558678607348, -288.5397485678157068, -271.3142857673570916 ) ) ;
#3017=CARTESIAN_POINT ( 'NONE',  ( -109.6645173009884076, -295.5112285779792956, -257.8494985183143058 ) ) ;
#3018=CARTESIAN_POINT ( 'NONE',  ( -69.31102360988489863, -287.6169388157089770, -337.3598331948587088 ) ) ;
#3019=CARTESIAN_POINT ( 'NONE',  ( 22.29632774050155319, -23.10002859818378340, -338.8215327972035311 ) ) ;
#3020=CARTESIAN_POINT ( 'NONE',  ( -98.04167817466826307, -293.9517282718423985, -314.4343059470606363 ) ) ;
#3021=CARTESIAN_POINT ( 'NONE',  ( 24.15608193541861581, -285.4265580190075298, -225.1866721606569115 ) ) ;
#3022=CARTESIAN_POINT ( 'NONE',  ( 30.05325989315680957, -283.5543187774048874, -300.5592469201921517 ) ) ;
#3023=CARTESIAN_POINT ( 'NONE',  ( -78.62819165778435604, -281.8398905386174533, -334.1529640879004432 ) ) ;
#3024=CARTESIAN_POINT ( 'NONE',  ( -63.82089453060896034, -289.4071338496478916, -338.4436225798462488 ) ) ;
#3025=CARTESIAN_POINT ( 'NONE',  ( 18.95676949748348150, -283.6453954953609582, -317.7711614054133520 ) ) ;
#3026=CARTESIAN_POINT ( 'NONE',  ( -36.18073762146470074, -283.8400618162410183, -343.5133831118960188 ) ) ;
#3027=CARTESIAN_POINT ( 'NONE',  ( 37.71393172772059899, -289.4391299682946510, -263.0903383623077616 ) ) ;
#3029=CARTESIAN_POINT ( 'NONE',  ( -26.21185907515926772, -298.3545741468140591, -193.3608124155709902 ) ) ;
#3031=CARTESIAN_POINT ( 'NONE',  ( -96.02768843728122761, -273.2243337611700440, -220.4914962255848536 ) ) ;
#3033=CARTESIAN_POINT ( 'NONE',  ( -44.48209383374271653, -293.9414057577958488, -196.0066536928164851 ) ) ;
#3035=CARTESIAN_POINT ( 'NONE',  ( -54.49178911615187815, -282.3376638359844719, -195.3683826091709363 ) ) ;
#3036=CARTESIAN_POINT ( 'NONE',  ( 37.55162405153379268, -273.6340407221134683, -276.7656802560686629 ) ) ;
#3037=DIRECTION ( 'NONE',  ( 0.000000000000000000, 0.000000000000000000, -1.000000000000000000 ) ) ;
#3038=CARTESIAN_POINT ( 'NONE',  ( -35.47558221234827158, -296.4750249970931009, -194.1616107217360252 ) ) ;
#3039=CARTESIAN_POINT ( 'NONE',  ( -110.2057400926187825, -291.9983672487444437, -282.1567865367271111 ) ) ;
#3040=CARTESIAN_POINT ( 'NONE',  ( -43.48242765931818354, -273.3212619719324721, -197.4667772659005891 ) ) ;
#3041=CARTESIAN_POINT ( 'NONE',  ( -106.3668036116438458, -292.4150927758277589, -244.4045357148850997 ) ) ;
#3042=CARTESIAN_POINT ( 'NONE',  ( -17.37993872388247141, -293.2572709366335744, -199.8460532097747091 ) ) ;
#3043=CARTESIAN_POINT ( 'NONE',  ( -76.64652642244364245, -285.3457353450075402, -333.1361879564246919 ) ) ;
#3044=CARTESIAN_POINT ( 'NONE',  ( -105.4869049485316168, -292.4271843175775416, -235.6779807014726771 ) ) ;
#3045=CARTESIAN_POINT ( 'NONE',  ( -58.81640960301491106, -293.0951848331761198, -196.9299588974726589 ) ) ;
#3046=CARTESIAN_POINT ( 'NONE',  ( -39.69116431654797594, -294.9157623180346377, -343.3357305434871591 ) ) ;
#3047=CARTESIAN_POINT ( 'NONE',  ( 15.51034928217692510, -290.3048975154570144, -323.5744764621534273 ) ) ;
#3048=CARTESIAN_POINT ( 'NONE',  ( 27.85022165064060218, -281.1811771619723572, -229.2854337535828222 ) ) ;
#3049=CARTESIAN_POINT ( 'NONE',  ( -51.50623766145860571, -295.9523515955251014, -196.0873153619806430 ) ) ;
#3050=CARTESIAN_POINT ( 'NONE',  ( -110.2253665077959823, -284.0725096859965220, -295.2000225387272394 ) ) ;
#3051=CARTESIAN_POINT ( 'NONE',  ( -3.090780735409602187, -278.5771951035954999, -336.6839747249878769 ) ) ;
#3052=CARTESIAN_POINT ( 'NONE',  ( -107.7772799113469091, -283.0749666145505330, -291.0448133529571351 ) ) ;
#3053=CARTESIAN_POINT ( 'NONE',  ( -13.31955261483823527, -284.3639863407584016, -199.3122821290266415 ) ) ;
#3054=CARTESIAN_POINT ( 'NONE',  ( -51.11174979524055573, -275.3659373070663037, -344.8640790656508557 ) ) ;
#3056=CARTESIAN_POINT ( 'NONE',  ( -2.404747239855777430, -282.0843592358984324, -334.5423710278622025 ) ) ;
#3057=CARTESIAN_POINT ( 'NONE',  ( -53.69077580166315045, -281.0520664835295293, -195.4688937955734502 ) ) ;
#3058=CARTESIAN_POINT ( 'NONE',  ( 21.91620773548717693, -285.9532751934067392, -221.5623416704565045 ) ) ;
#3059=CARTESIAN_POINT ( 'NONE',  ( 34.10064247204049082, -295.5648138790134567, -289.7475538954539047 ) ) ;
#3060=CARTESIAN_POINT ( 'NONE',  ( 22.89826290227155781, -277.7821046158716172, -317.0469120987233396 ) ) ;
#3061=CARTESIAN_POINT ( 'NONE',  ( 38.00350234478532485, -276.6992061323920780, -257.0048325610704865 ) ) ;
#3062=CARTESIAN_POINT ( 'NONE',  ( -80.82108114090546280, -277.4944608506777399, -329.0002127165847128 ) ) ;
#3063=CARTESIAN_POINT ( 'NONE',  ( -66.30523341228550294, -299.6722401642571185, -201.3600877877883022 ) ) ;
#3064=CARTESIAN_POINT ( 'NONE',  ( -1.281123231060983469, -284.5310798975464195, -204.7311511825882349 ) ) ;
#3065=CARTESIAN_POINT ( 'NONE',  ( -108.7315755454474697, -292.4944906565732481, -243.5662014241347038 ) ) ;
#3066=CARTESIAN_POINT ( 'NONE',  ( 0.07860816415507965171, -291.4833429118256731, -207.3218714691700484 ) ) ;
#3068=CARTESIAN_POINT ( 'NONE',  ( -14.83585392158876459, -292.0186628350635942, -200.8947637292160948 ) ) ;
#3070=CARTESIAN_POINT ( 'NONE',  ( 14.40531861230846467, -289.4246479270315149, -327.0346702897856517 ) ) ;
#3071=CARTESIAN_POINT ( 'NONE',  ( -57.14878627495813390, -280.4411715149433917, -199.9937107100818139 ) ) ;
#3073=CARTESIAN_POINT ( 'NONE',  ( -112.8324078728765301, -295.6421855100037419, -256.8464757572042458 ) ) ;
#3074=CARTESIAN_POINT ( 'NONE',  ( 16.62034589414837171, -288.9607096590137303, -325.2203012307290919 ) ) ;
#3075=CARTESIAN_POINT ( 'NONE',  ( 28.67822697776172447, -287.3678649460407541, -230.6715384530783695 ) ) ;
#3076=CARTESIAN_POINT ( 'NONE',  ( -91.67794081615380719, -284.1872729663721771, -319.1616948540911949 ) ) ;
#3077=CARTESIAN_POINT ( 'NONE',  ( 201.8898544361462939, 293.7279171300682492, -83.20153124629544550 ) ) ;
#3078=CARTESIAN_POINT ( 'NONE',  ( -91.05905222517534980, -229.2228000228819553, -346.3972628765899913 ) ) ;
#3079=CARTESIAN_POINT ( 'NONE',  ( 172.7241459038852724, 240.9461585357967977, -177.0720788202972642 ) ) ;
#3080=CARTESIAN_POINT ( 'NONE',  ( -40.52299827980939284, -276.2903069137316834, -343.4658875544013199 ) ) ;
#3081=CARTESIAN_POINT ( 'NONE',  ( -69.39895019544928800, -276.4044892244371567, -336.3034515216097589 ) ) ;
#3082=CARTESIAN_POINT ( 'NONE',  ( -68.83153142094452903, -273.3161080052328202, -200.1033302448623488 ) ) ;
#3083=CARTESIAN_POINT ( 'NONE',  ( 168.8266546690683469, 229.6582186635458811, -190.4167746751373045 ) ) ;
#3084=CARTESIAN_POINT ( 'NONE',  ( -12.04514565589438391, -275.4146594927864271, -342.6204389095458964 ) ) ;
#3086=CARTESIAN_POINT ( 'NONE',  ( -45.36298306592939866, -289.6488715600345927, -342.9810013592488076 ) ) ;
#3087=CARTESIAN_POINT ( 'NONE',  ( -97.22694137413476767, -298.0015441995196852, -222.2163705817446555 ) ) ;
#3088=CARTESIAN_POINT ( 'NONE',  ( -110.7392032743995856, -296.7538416112298023, -293.4775556820247857 ) ) ;
#3089=CARTESIAN_POINT ( 'NONE',  ( -77.94797901830229137, -295.7810334968511938, -331.0862488517759630 ) ) ;
#3091=CARTESIAN_POINT ( 'NONE',  ( -98.47012575264064083, -279.8715112114314252, -314.7974066838259546 ) ) ;
#3093=CARTESIAN_POINT ( 'NONE',  ( 2.057236658432576526, -282.0471212020546545, -336.4462954681184215 ) ) ;
#3094=CARTESIAN_POINT ( 'NONE',  ( -95.86679617888430016, -280.2495778382210005, -226.1923521755928448 ) ) ;
#3095=CARTESIAN_POINT ( 'NONE',  ( 18.17832909697120769, -278.0292572741548724, -322.2407899997566005 ) ) ;
#3097=CARTESIAN_POINT ( 'NONE',  ( -75.50078601134499934, -296.1074769172285528, -207.3794021907888805 ) ) ;
#3099=CARTESIAN_POINT ( 'NONE',  ( -92.20984144269753813, -279.4062738393386098, -222.1914310669604049 ) ) ;
#3100=CARTESIAN_POINT ( 'NONE',  ( -58.08786774099759498, -274.5936933841057339, -196.3209753106200992 ) ) ;
#3101=CARTESIAN_POINT ( 'NONE',  ( 29.92109096748625419, -286.7128903450975486, -306.9275318989845118 ) ) ;
#3102=CARTESIAN_POINT ( 'NONE',  ( -97.96586353315110784, -275.1549477435995072, -226.1194276546539186 ) ) ;
#3103=CARTESIAN_POINT ( 'NONE',  ( 33.63017435991903170, -274.4904678438071528, -298.8162146314662095 ) ) ;
#3105=CARTESIAN_POINT ( 'NONE',  ( -80.51101045638458231, -288.8511520479362389, -329.4920280820580842 ) ) ;
#3106=CARTESIAN_POINT ( 'NONE',  ( -112.4273608584512658, -283.6929006306159522, -286.9579953948043567 ) ) ;
#3107=CARTESIAN_POINT ( 'NONE',  ( -5.618676244901598338, -280.8690342811481173, -337.2452585550860249 ) ) ;
#3108=CARTESIAN_POINT ( 'NONE',  ( 36.15349400680588587, -280.1755402659749734, -274.0801709193741544 ) ) ;
#3109=CARTESIAN_POINT ( 'NONE',  ( -57.76646952932928514, -283.8663224293867415, -198.7243532075731309 ) ) ;
#3110=CARTESIAN_POINT ( 'NONE',  ( -70.07719201519769570, -291.4834696180043920, -337.8539023633189800 ) ) ;
#3111=CARTESIAN_POINT ( 'NONE',  ( -99.81372407934746604, -280.2867524017653409, -231.7365177741657192 ) ) ;
#3112=CARTESIAN_POINT ( 'NONE',  ( -103.8239762884536503, -271.0130733266666994, -235.5342847911063302 ) ) ;
#3113=CARTESIAN_POINT ( 'NONE',  ( -27.49587067370445581, -281.3290688088525258, -345.9751576346699267 ) ) ;
#3114=CARTESIAN_POINT ( 'NONE',  ( 36.09817803515041135, -295.3561070683542766, -255.0803593480729319 ) ) ;
#3115=CARTESIAN_POINT ( 'NONE',  ( -31.13389149590402738, -278.3692832688519729, -194.5764519779699526 ) ) ;
#3116=CARTESIAN_POINT ( 'NONE',  ( -108.5837353612852354, -278.9869936502050223, -286.8014701598497140 ) ) ;
#3117=CARTESIAN_POINT ( 'NONE',  ( -24.81345774986261787, -284.8929889093944894, -344.5292069607254462 ) ) ;
#3118=EDGE_CURVE ( 'NONE', #10505, #31408, #2105, .T. ) ;
#3120=PLANE ( 'NONE',  #65582 ) ;
#3121=CARTESIAN_POINT ( 'NONE',  ( -63.90589228720160264, -293.6287176404612751, -199.5694485526131814 ) ) ;
#3122=CARTESIAN_POINT ( 'NONE',  ( 36.67689324420568653, -273.7112893889893144, -282.7676018470114627 ) ) ;
#3123=CARTESIAN_POINT ( 'NONE',  ( 39.47883557998053305, -286.7284846699095624, -268.6985556441270546 ) ) ;
#3124=CARTESIAN_POINT ( 'NONE',  ( -55.18628355259232166, -290.2186476542224227, -198.7509842342544744 ) ) ;
#3126=CARTESIAN_POINT ( 'NONE',  ( 32.56211506881474804, -274.5359562479713986, -293.0481208463745020 ) ) ;
#3127=CARTESIAN_POINT ( 'NONE',  ( -61.43610201560318274, -293.5078943124126454, -340.6318805672689791 ) ) ;
#3128=DIRECTION ( 'NONE',  ( 0.9951408606192333473, 0.000000000000000000, -0.09846150276129089773 ) ) ;
#3130=CARTESIAN_POINT ( 'NONE',  ( 38.80879532418298794, -292.1032865527982381, -276.0073016608375838 ) ) ;
#3131=CARTESIAN_POINT ( 'NONE',  ( -35.93846714110579654, -287.6701726972185611, -196.5744568950748317 ) ) ;
#3132=CARTESIAN_POINT ( 'NONE',  ( -12.57546657330419393, -286.9744693794624482, -342.2536172055258135 ) ) ;
#3133=CARTESIAN_POINT ( 'NONE',  ( 13.53391193484293353, -288.2064127064416539, -217.1208506087276646 ) ) ;
#3135=CARTESIAN_POINT ( 'NONE',  ( 34.44458160300596461, -288.5416754317006962, -284.5444050319245548 ) ) ;
#3136=CARTESIAN_POINT ( 'NONE',  ( 31.80490320440512875, -295.1420089349788327, -240.4085880801197845 ) ) ;
#3138=CARTESIAN_POINT ( 'NONE',  ( 39.18007486906842018, -288.7002209067438230, -265.8265251596110943 ) ) ;
#3139=CARTESIAN_POINT ( 'NONE',  ( -53.84108145133048851, -275.3420229753857598, -344.1513293236438926 ) ) ;
#3140=CARTESIAN_POINT ( 'NONE',  ( -102.0769076686427894, -278.3376488508054081, -312.1128748316036194 ) ) ;
#3141=CARTESIAN_POINT ( 'NONE',  ( 20.11573350605875277, -280.5239699987596396, -219.1125193097255703 ) ) ;
#3142=CARTESIAN_POINT ( 'NONE',  ( -58.39224187424481016, -299.7585883280645476, -198.7460253527467842 ) ) ;
#3144=CARTESIAN_POINT ( 'NONE',  ( -44.18210449760081104, -283.9654691773182549, -195.6737059470788722 ) ) ;
#3146=CARTESIAN_POINT ( 'NONE',  ( -101.6647520232515660, -276.1908534411145411, -307.5239685529722351 ) ) ;
#3147=CARTESIAN_POINT ( 'NONE',  ( 37.64219235886115200, -279.5109957541901622, -267.1685931404740018 ) ) ;
#3149=CARTESIAN_POINT ( 'NONE',  ( -38.55353751901358805, -275.5469734511579531, -346.6581638315258260 ) ) ;
#3150=CARTESIAN_POINT ( 'NONE',  ( -106.6325460656534574, -297.7394181985087016, -295.6006231813223053 ) ) ;
#3151=CARTESIAN_POINT ( 'NONE',  ( -4.309480011362734508, -281.5472517469743821, -339.5880098019582078 ) ) ;
#3152=CARTESIAN_POINT ( 'NONE',  ( -103.9375315631847059, -297.9044591093028771, -239.7692950969522485 ) ) ;
#3153=CARTESIAN_POINT ( 'NONE',  ( -87.15395982469463831, -298.6905374437307614, -212.2220226413342061 ) ) ;
#3154=CARTESIAN_POINT ( 'NONE',  ( 19.87471900312880990, -274.5784544573400581, -224.9718588033083506 ) ) ;
#3155=CARTESIAN_POINT ( 'NONE',  ( 36.81942298719200579, -295.7002883529291353, -281.8857563062040867 ) ) ;
#3156=CARTESIAN_POINT ( 'NONE',  ( 37.71915334566357103, -287.5034156985354343, -253.1308786954831191 ) ) ;
#3157=CARTESIAN_POINT ( 'NONE',  ( -98.25228059568989636, -277.2374212787451597, -225.6267039745527256 ) ) ;
#3158=CARTESIAN_POINT ( 'NONE',  ( -112.5657980065144983, -290.1798448089752469, -286.8029884026397553 ) ) ;
#3159=CARTESIAN_POINT ( 'NONE',  ( 17.96171838373200558, -285.9286965936914271, -222.3513236743515620 ) ) ;
#3160=CARTESIAN_POINT ( 'NONE',  ( -6.680634681508814232, -290.4544925771463681, -201.9008708072903744 ) ) ;
#3162=CARTESIAN_POINT ( 'NONE',  ( 23.55732936118107901, -287.6197140082176134, -310.7485135007678991 ) ) ;
#3164=CARTESIAN_POINT ( 'NONE',  ( -99.16190811959243945, -286.1008385486072143, -224.7644959229374990 ) ) ;
#3165=CARTESIAN_POINT ( 'NONE',  ( -2.152982846972653075, -291.5651546628753863, -202.1219432100804170 ) ) ;
#3166=CARTESIAN_POINT ( 'NONE',  ( 27.16316385631357022, -282.6143944792402749, -229.6967351381213405 ) ) ;
#3167=CARTESIAN_POINT ( 'NONE',  ( -17.13843939398215710, -281.6228536193876266, -196.5700173861686721 ) ) ;
#3169=CARTESIAN_POINT ( 'NONE',  ( -67.78630364169399058, -283.2965420665266834, -336.7096380974146541 ) ) ;
#3170=CARTESIAN_POINT ( 'NONE',  ( -113.6526282743976708, -296.4187247969506416, -281.0298623535917955 ) ) ;
#3171=CARTESIAN_POINT ( 'NONE',  ( -85.64682327319778210, -274.6826751743233785, -214.9050234370071450 ) ) ;
#3172=CARTESIAN_POINT ( 'NONE',  ( 34.90641323735309243, -291.3300079090541317, -251.5979380625179544 ) ) ;
#3173=CARTESIAN_POINT ( 'NONE',  ( -21.83525760534138627, -273.0502545481738821, -198.6207475910898097 ) ) ;
#3176=CARTESIAN_POINT ( 'NONE',  ( -74.49469757111489798, -285.4701770953417395, -334.9254219910689017 ) ) ;
#3177=CARTESIAN_POINT ( 'NONE',  ( -22.14529752142060204, -295.9415392033025114, -345.5313371967322951 ) ) ;
#3178=CARTESIAN_POINT ( 'NONE',  ( -97.61169086423342378, -284.6274329276824346, -311.8186506267267077 ) ) ;
#3179=CARTESIAN_POINT ( 'NONE',  ( -7.985738926497114143, -275.7356267870846978, -341.3052370359391148 ) ) ;
#3180=CARTESIAN_POINT ( 'NONE',  ( 39.55375964649560672, -294.1668854424063966, -267.4321988208715197 ) ) ;
#3181=CARTESIAN_POINT ( 'NONE',  ( 24.54999461602020006, -285.1037932265534209, -226.6383561968136462 ) ) ;
#3182=CARTESIAN_POINT ( 'NONE',  ( 24.79487604314860860, -293.2819738738166393, -224.9211554682974565 ) ) ;
#3183=CARTESIAN_POINT ( 'NONE',  ( -98.85729388595689215, -290.3413811284460735, -309.7047224357694972 ) ) ;
#3185=DIRECTION ( 'NONE',  ( 0.000000000000000000, 0.000000000000000000, -1.000000000000000000 ) ) ;
#3186=CARTESIAN_POINT ( 'NONE',  ( 84.93309205534008299, 81.36957093815985331, -298.8374046425330448 ) ) ;
#3187=CARTESIAN_POINT ( 'NONE',  ( -103.8035332550911392, -285.5801295624835916, -307.9585234203994446 ) ) ;
#3188=CARTESIAN_POINT ( 'NONE',  ( 25.22466315766302358, -278.4094976428775681, -220.5068182859052968 ) ) ;
#3190=CARTESIAN_POINT ( 'NONE',  ( -38.90540172793681251, -281.9925159454898562, -343.6660957841280037 ) ) ;
#3191=CARTESIAN_POINT ( 'NONE',  ( -77.80739894272457491, -277.2462581844129090, -335.9079588489759658 ) ) ;
#3192=CARTESIAN_POINT ( 'NONE',  ( -4.783303107571053481, -282.4821269198680511, -202.9817501106678321 ) ) ;
#3193=CARTESIAN_POINT ( 'NONE',  ( 86.54078617439742516, 81.51664523006699881, -300.9066486022009599 ) ) ;
#3194=CARTESIAN_POINT ( 'NONE',  ( 8.838160785872977598, -281.0073569661338411, -331.2382626041874687 ) ) ;
#3195=CARTESIAN_POINT ( 'NONE',  ( 37.29967594461567870, -285.5814833268626671, -271.0765042700479057 ) ) ;
#3196=CARTESIAN_POINT ( 'NONE',  ( -32.02081407409072256, -299.8780319020539196, -194.3728757402488441 ) ) ;
#3197=CARTESIAN_POINT ( 'NONE',  ( -75.68501931998575571, -296.0709155532713908, -332.6115627939650494 ) ) ;
#3199=CARTESIAN_POINT ( 'NONE',  ( 23.76049941203009652, -291.6736650922729837, -229.5228431721685922 ) ) ;
#3200=CARTESIAN_POINT ( 'NONE',  ( -112.3042237070368969, -279.4182610784516783, -253.2166481482915970 ) ) ;
#3201=CARTESIAN_POINT ( 'NONE',  ( 9.485080266334289689, -274.7168091038886928, -214.2926665229085756 ) ) ;
#3202=CARTESIAN_POINT ( 'NONE',  ( 29.68409321610350560, -273.9862011148551915, -232.9821150870422457 ) ) ;
#3203=DIRECTION ( 'NONE',  ( -1.000000000000000000, -0.000000000000000000, -0.000000000000000000 ) ) ;
#3204=CARTESIAN_POINT ( 'NONE',  ( 11.87504125697724611, -272.7353163065756121, -213.7007498005672232 ) ) ;
#3205=CARTESIAN_POINT ( 'NONE',  ( 21.84186392373628749, -295.6313442226972938, -318.7129388050902890 ) ) ;
#3208=CARTESIAN_POINT ( 'NONE',  ( -109.9201869115441781, -285.7674474160023692, -260.0369071200122448 ) ) ;
#3209=CARTESIAN_POINT ( 'NONE',  ( 35.20154015585742968, -283.0243865427275409, -247.7458067330712197 ) ) ;
#3210=CARTESIAN_POINT ( 'NONE',  ( -76.18830825081796831, -282.9345695676315700, -332.3470213345502202 ) ) ;
#3211=CARTESIAN_POINT ( 'NONE',  ( -51.45359808223236797, -275.6354948520724406, -342.7993313043730836 ) ) ;
#3212=CARTESIAN_POINT ( 'NONE',  ( 31.48851192887348205, -283.7787441181668555, -298.1688037236652917 ) ) ;
#3213=CARTESIAN_POINT ( 'NONE',  ( -36.47728199580403441, -275.5210373603086964, -344.0619698814880962 ) ) ;
#3214=CARTESIAN_POINT ( 'NONE',  ( 13.70207272223562178, -275.8679550096711637, -217.7421164110424172 ) ) ;
#3217=CARTESIAN_POINT ( 'NONE',  ( -31.09709954890292494, -280.9318436103359886, -193.7241804183869931 ) ) ;
#3218=CARTESIAN_POINT ( 'NONE',  ( 20.07857662489317008, -281.3494650320590722, -219.1315579260468382 ) ) ;
#3221=CARTESIAN_POINT ( 'NONE',  ( -15.78790135731870947, -288.1883546324197596, -197.6723359921274437 ) ) ;
#3222=CARTESIAN_POINT ( 'NONE',  ( -37.00505171732093856, -294.2449637719207658, -343.5342719649205492 ) ) ;
#3223=CARTESIAN_POINT ( 'NONE',  ( -113.2607411498891281, -289.7475656991182973, -282.5927162835344006 ) ) ;
#3224=CARTESIAN_POINT ( 'NONE',  ( 34.37596487510375454, -285.5532896977239261, -252.0191782791793003 ) ) ;
#3225=CARTESIAN_POINT ( 'NONE',  ( 36.21814932527016850, -286.1719439005656795, -273.8053620493907943 ) ) ;
#3226=CARTESIAN_POINT ( 'NONE',  ( -57.91541754910730333, -290.0227392740632126, -199.2111255646440213 ) ) ;
#3227=CARTESIAN_POINT ( 'NONE',  ( -22.39388310276886429, -287.4527762011890104, -198.4501148162585196 ) ) ;
#3228=CARTESIAN_POINT ( 'NONE',  ( -83.65198204334981824, -275.6869242687699284, -329.4216884099090521 ) ) ;
#3229=CARTESIAN_POINT ( 'NONE',  ( 32.12710830490041758, -286.3562172689345289, -301.6744548911016182 ) ) ;
#3230=CARTESIAN_POINT ( 'NONE',  ( -18.70430708143557652, -288.2921875845780733, -197.6600272521977786 ) ) ;
#3231=CARTESIAN_POINT ( 'NONE',  ( 37.74772135464480272, -285.4955006648787617, -265.9519459777102384 ) ) ;
#3232=CARTESIAN_POINT ( 'NONE',  ( 35.37489605523790459, -282.6132585092693716, -279.4756645447856727 ) ) ;
#3233=CARTESIAN_POINT ( 'NONE',  ( -0.1647487453744717611, -290.5593828577046907, -335.7491328647454907 ) ) ;
#3237=CARTESIAN_POINT ( 'NONE',  ( -112.9250856760444748, -298.4456253468944169, -272.4547568002766411 ) ) ;
#3238=CARTESIAN_POINT ( 'NONE',  ( 33.88377705627229375, -279.2465434819816323, -246.7040258299916218 ) ) ;
#3239=CARTESIAN_POINT ( 'NONE',  ( -47.71145770650421269, -291.1208084651235026, -194.1718542637828762 ) ) ;
#3240=CARTESIAN_POINT ( 'NONE',  ( -92.80522687419166061, -294.2646205408400419, -319.0462041717752300 ) ) ;
#3241=CARTESIAN_POINT ( 'NONE',  ( 11.64691924035343717, -279.4341169229158481, -215.5764609222925685 ) ) ;
#3242=CARTESIAN_POINT ( 'NONE',  ( -67.62128913285192766, -271.7316188445224157, -202.3437700395113268 ) ) ;
#3243=CARTESIAN_POINT ( 'NONE',  ( -68.71273156986022457, -296.7884836583860988, -336.8362218243789812 ) ) ;
#3244=CARTESIAN_POINT ( 'NONE',  ( -95.56682381678963623, -271.7992918970323899, -220.8592517632580723 ) ) ;
#3245=CARTESIAN_POINT ( 'NONE',  ( 8.279646956727130913, -292.6772831150340721, -331.1284340458325346 ) ) ;
#3246=CARTESIAN_POINT ( 'NONE',  ( -0.9812017884011294822, -293.9701704699788252, -206.3677102599160946 ) ) ;
#3248=CARTESIAN_POINT ( 'NONE',  ( 32.78091438322449136, -294.0773592550401645, -249.3198927158008473 ) ) ;
#3250=FACE_BOUND ( 'NONE', #1362, .T. ) ;
#3251=CARTESIAN_POINT ( 'NONE',  ( -94.11255491464412160, -281.8875079250580029, -319.9138863375851543 ) ) ;
#3252=CARTESIAN_POINT ( 'NONE',  ( -41.03921944085710294, -295.0999438261267755, -343.2799837038897977 ) ) ;
#3253=CARTESIAN_POINT ( 'NONE',  ( 22.52326512964628336, -282.2017200253790747, -318.8090409811625818 ) ) ;
#3254=CARTESIAN_POINT ( 'NONE',  ( -22.86645706011551127, -282.1559836653042908, -196.1473679702848187 ) ) ;
#3255=CARTESIAN_POINT ( 'NONE',  ( -7.347449989516855240, -286.1014655196306649, -199.4095594324957688 ) ) ;
#3256=CARTESIAN_POINT ( 'NONE',  ( -111.6121051130163693, -288.4340928879395847, -279.5227427972042733 ) ) ;
#3257=CARTESIAN_POINT ( 'NONE',  ( -30.29833455534296860, -281.4444596772003138, -346.3420284385918535 ) ) ;
#3258=CARTESIAN_POINT ( 'NONE',  ( 5.373708009634825089, -287.4089358795773705, -334.0548101093624496 ) ) ;
#3260=CARTESIAN_POINT ( 'NONE',  ( -89.04797160909069476, -297.3936470175174236, -323.0912663003654757 ) ) ;
#3261=CARTESIAN_POINT ( 'NONE',  ( 37.02265668121343367, -277.1994463476847841, -287.9830897149314524 ) ) ;
#3262=CARTESIAN_POINT ( 'NONE',  ( 37.59847648380248586, -291.6793053756771883, -278.7376271320996466 ) ) ;
#3263=CARTESIAN_POINT ( 'NONE',  ( -107.6375145660343691, -278.4805832761761621, -250.5515366300710127 ) ) ;
#3264=CARTESIAN_POINT ( 'NONE',  ( 38.32484388043344126, -293.5403911187398762, -256.0931776150931682 ) ) ;
#3265=CARTESIAN_POINT ( 'NONE',  ( -75.36061662161361596, -283.6296659964604601, -205.0025134999579564 ) ) ;
#3266=CARTESIAN_POINT ( 'NONE',  ( -56.39080640651074106, -279.2976468192235870, -342.9552907756294644 ) ) ;
#3267=CARTESIAN_POINT ( 'NONE',  ( -1.129938079112184912, -291.6040282042743002, -206.6903560878875226 ) ) ;
#3268=CARTESIAN_POINT ( 'NONE',  ( -99.67364875471277230, -271.1200460979784452, -228.2594931903377073 ) ) ;
#3271=CARTESIAN_POINT ( 'NONE',  ( 33.36934294880997243, -292.8173123691423143, -251.9780597820586650 ) ) ;
#3273=CARTESIAN_POINT ( 'NONE',  ( -6.998514795304330072, -286.1237833571631768, -333.4427485647536855 ) ) ;
#3274=CARTESIAN_POINT ( 'NONE',  ( -33.33765991442466259, -297.1598859787685569, -193.5970321323677865 ) ) ;
#3275=CARTESIAN_POINT ( 'NONE',  ( -35.17906740486936457, -287.3939084084247497, -193.8717792726471600 ) ) ;
#3276=CARTESIAN_POINT ( 'NONE',  ( 30.48439716770303676, -287.7482690112159958, -297.4904141672690230 ) ) ;
#3277=CARTESIAN_POINT ( 'NONE',  ( -103.7474611906482949, -279.6426332942239128, -302.4319490299551489 ) ) ;
#3278=CARTESIAN_POINT ( 'NONE',  ( -84.74074546509368133, -299.1489603889610294, -213.4496210277129933 ) ) ;
#3279=CARTESIAN_POINT ( 'NONE',  ( -39.69869221830266781, -278.8168503100827138, -196.9893103965865748 ) ) ;
#3280=EDGE_LOOP ( 'NONE', ( #62154, #23611, #77651, #73879 ) ) ;
#3281=CARTESIAN_POINT ( 'NONE',  ( -9.115682335510763679, -298.0632170819999374, -193.3838024440057382 ) ) ;
#3282=CARTESIAN_POINT ( 'NONE',  ( -0.5661350211931107657, -294.4649723526099478, -205.6248638718004145 ) ) ;
#3283=CARTESIAN_POINT ( 'NONE',  ( 32.58212755522404080, -294.7623062535610643, -240.0774798978839613 ) ) ;
#3285=CARTESIAN_POINT ( 'NONE',  ( -98.92317465171700519, -290.6594618712950933, -309.7516582634343081 ) ) ;
#3287=CARTESIAN_POINT ( 'NONE',  ( 28.41554031329198082, -291.1948374564298661, -232.7274786695991793 ) ) ;
#3289=CARTESIAN_POINT ( 'NONE',  ( -72.85345360504487644, -297.2344932337986734, -206.5567070707547828 ) ) ;
#3292=CARTESIAN_POINT ( 'NONE',  ( -110.8686674365253282, -291.8142579168338671, -290.7692740041106845 ) ) ;
#3293=CARTESIAN_POINT ( 'NONE',  ( 36.60358173371528068, -290.4805209788416391, -305.9350535429201159 ) ) ;
#3294=CARTESIAN_POINT ( 'NONE',  ( -37.30491739858693734, -288.0527346028062539, -195.5150379833580416 ) ) ;
#3295=CARTESIAN_POINT ( 'NONE',  ( -13.45676503978470251, -272.3628528579907311, -199.4418801069632252 ) ) ;
#3296=CARTESIAN_POINT ( 'NONE',  ( 1.340272797033512653, -276.4934163097516375, -206.7606528268024135 ) ) ;
#3298=CARTESIAN_POINT ( 'NONE',  ( 22.15926449107730534, -291.0160333956610543, -225.6291449652785275 ) ) ;
#3299=CARTESIAN_POINT ( 'NONE',  ( -77.14549112972787270, -279.4396016717453790, -334.8888388176876560 ) ) ;
#3301=CARTESIAN_POINT ( 'NONE',  ( -69.06088858312446632, -282.8292890359639955, -336.2368098477783178 ) ) ;
#3302=CARTESIAN_POINT ( 'NONE',  ( -94.96939602140655268, -278.9442615027691659, -320.9629082307384920 ) ) ;
#3304=CARTESIAN_POINT ( 'NONE',  ( 37.86777583068692365, -280.1642391187898511, -255.8165847958368033 ) ) ;
#3305=CARTESIAN_POINT ( 'NONE',  ( -64.37108594678602458, -181.9596566217732914, -359.3138851375881586 ) ) ;
#3306=CARTESIAN_POINT ( 'NONE',  ( 39.38880183194059725, -276.5393117308727824, -274.0207565710887820 ) ) ;
#3308=CARTESIAN_POINT ( 'NONE',  ( -4.145390490588479082, -276.0020011739800907, -201.6392988562928679 ) ) ;
#3309=CARTESIAN_POINT ( 'NONE',  ( -69.85430415644619018, -297.9805209788416391, -337.9475929042657754 ) ) ;
#3313=CARTESIAN_POINT ( 'NONE',  ( -70.09826347096063159, -290.5738688192431596, -335.9588250696023124 ) ) ;
#3314=CARTESIAN_POINT ( 'NONE',  ( -41.68000079072222519, -290.8662038289725160, -346.2368919982716307 ) ) ;
#3315=CARTESIAN_POINT ( 'NONE',  ( -109.3757603311664184, -290.0685400739879469, -257.6229172631110487 ) ) ;
#3316=CARTESIAN_POINT ( 'NONE',  ( 9.778015517621573949, -286.1891212163698128, -209.5395814965136196 ) ) ;
#3318=CARTESIAN_POINT ( 'NONE',  ( 30.03661558084898786, -280.3545769650451689, -300.5963633306288898 ) ) ;
#3319=CARTESIAN_POINT ( 'NONE',  ( 24.55222554496365106, -289.9720976208146794, -311.3722411185597139 ) ) ;
#3320=CARTESIAN_POINT ( 'NONE',  ( -45.73750329682886218, -281.6402312371427001, -343.6261088063008629 ) ) ;
#3321=CARTESIAN_POINT ( 'NONE',  ( 34.71750494821791477, -283.0574604377915762, -284.8714733654586553 ) ) ;
#3322=CARTESIAN_POINT ( 'NONE',  ( 39.46722419409472593, -288.5081374216714494, -271.5356888175278982 ) ) ;
#3323=CARTESIAN_POINT ( 'NONE',  ( -108.3509578115677812, -279.2711797265430391, -253.1659510713735131 ) ) ;
#3324=CARTESIAN_POINT ( 'NONE',  ( -98.02425376813560831, -289.9744038353175597, -223.5891087115241191 ) ) ;
#3325=CARTESIAN_POINT ( 'NONE',  ( -57.72296622173877267, -286.5984343889253978, -196.2196953537114723 ) ) ;
#3326=CARTESIAN_POINT ( 'NONE',  ( 24.64996416893101738, -287.4387019231546105, -224.7918250204139099 ) ) ;
#3327=CARTESIAN_POINT ( 'NONE',  ( -104.1124439977133562, -284.3217342683776110, -299.8681979394119708 ) ) ;
#3330=CARTESIAN_POINT ( 'NONE',  ( -3.888440784880806689, -294.3490796603538797, -202.3675184288472053 ) ) ;
#3331=CARTESIAN_POINT ( 'NONE',  ( 36.94713547685543631, -292.0067257337372553, -252.0726741169643788 ) ) ;
#3332=CARTESIAN_POINT ( 'NONE',  ( 31.47876952186530630, -274.9452595870853884, -295.5514066198417140 ) ) ;
#3333=ADVANCED_FACE ( 'NONE', ( #83643 ), #32309, .T. ) ;
#3334=CARTESIAN_POINT ( 'NONE',  ( -24.93244843925003806, -294.2465778989452474, -346.3053164935913060 ) ) ;
#3335=CARTESIAN_POINT ( 'NONE',  ( -109.0981875987010739, -289.2520776972204999, -253.5218018858991798 ) ) ;
#3336=CARTESIAN_POINT ( 'NONE',  ( 18.72559985069543842, -292.4709175641842194, -318.6963935335374458 ) ) ;
#3337=CARTESIAN_POINT ( 'NONE',  ( -91.06020840915365966, -292.4726279651912932, -220.3280093818309240 ) ) ;
#3339=CARTESIAN_POINT ( 'NONE',  ( 23.34960531646590098, -290.9489093174582877, -226.0148230720368474 ) ) ;
#3340=CARTESIAN_POINT ( 'NONE',  ( 7.105927811645549319, -296.4473943804986789, -330.8352197173951481 ) ) ;
#3341=CARTESIAN_POINT ( 'NONE',  ( -15.77094140479450068, -289.7075302732210389, -340.4006211466099217 ) ) ;
#3342=CARTESIAN_POINT ( 'NONE',  ( 23.06459478745229319, -278.1443693137554192, -315.4109386283270169 ) ) ;
#3343=CARTESIAN_POINT ( 'NONE',  ( -37.14348105266689970, -275.8446178746968940, -346.9767815062695604 ) ) ;
#3344=CARTESIAN_POINT ( 'NONE',  ( -67.48802892612940241, -273.0155328330564544, -199.6185448967968625 ) ) ;
#3345=CARTESIAN_POINT ( 'NONE',  ( -49.35059724476386833, -277.9777276013978735, -196.8961563645111426 ) ) ;
#3346=CARTESIAN_POINT ( 'NONE',  ( -23.10852334831740862, -275.2730393374979485, -345.2736523688169541 ) ) ;
#3348=CARTESIAN_POINT ( 'NONE',  ( -108.0820080083184394, -294.9753395334382731, -290.2872897124192946 ) ) ;
#3349=CARTESIAN_POINT ( 'NONE',  ( 144.7857639756989272, -299.5541904835127980, -195.3611179825600175 ) ) ;
#3350=CARTESIAN_POINT ( 'NONE',  ( -62.07197012466863839, -274.3733237499686197, -201.5693567460409668 ) ) ;
#3353=CARTESIAN_POINT ( 'NONE',  ( -15.45460456147322859, -286.7904845927549218, -342.5222730165527310 ) ) ;
#3354=CARTESIAN_POINT ( 'NONE',  ( -24.59434719683853743, -274.0525546230624059, -198.4311249685764267 ) ) ;
#3356=CARTESIAN_POINT ( 'NONE',  ( 30.36269043639126508, -288.0278526685917768, -307.1484451448854429 ) ) ;
#3357=CARTESIAN_POINT ( 'NONE',  ( -9.884553245675764543, -300.3741332763799505, -194.9966984203866218 ) ) ;
#3358=CARTESIAN_POINT ( 'NONE',  ( -97.90682274181324374, -293.9517282735380377, -314.3363195487081043 ) ) ;
#3360=CARTESIAN_POINT ( 'NONE',  ( -66.52441117905529211, -282.6219065637503718, -341.4564131871359791 ) ) ;
#3363=CARTESIAN_POINT ( 'NONE',  ( -112.2859399133422329, -276.5005673606524965, -274.3658439002661567 ) ) ;
#3365=CARTESIAN_POINT ( 'NONE',  ( -107.3759221028292785, -289.6370752132515918, -248.3566074674033644 ) ) ;
#3369=CARTESIAN_POINT ( 'NONE',  ( -67.34130092343009721, -289.6585701269480637, -201.6223035945419042 ) ) ;
#3370=CARTESIAN_POINT ( 'NONE',  ( -49.00406835077139789, -275.4211536965879645, -197.5447889531275791 ) ) ;
#3371=CARTESIAN_POINT ( 'NONE',  ( 29.25731011628556999, -283.4683831290116700, -307.9280178847054117 ) ) ;
#3372=CARTESIAN_POINT ( 'NONE',  ( -77.30828217564319971, -295.5390933722094360, -206.4777937018711782 ) ) ;
#3373=CARTESIAN_POINT ( 'NONE',  ( -104.1132998724246619, -284.1550810543499779, -299.8662610525607874 ) ) ;
#3374=CARTESIAN_POINT ( 'NONE',  ( -38.10654969369583256, -275.4676571440381849, -196.7758618226220619 ) ) ;
#3375=CARTESIAN_POINT ( 'NONE',  ( 31.26620542559711069, -276.0169261289804581, -244.9533037860313129 ) ) ;
#3376=CARTESIAN_POINT ( 'NONE',  ( -8.776404072727224559, -284.6787398149948558, -339.7633288188958431 ) ) ;
#3379=CARTESIAN_POINT ( 'NONE',  ( 0.5386532627527429451, -294.3950790960922745, -337.4141883416912719 ) ) ;
#3380=CARTESIAN_POINT ( 'NONE',  ( -111.5039782348854089, -286.4169941999679168, -279.2793477202540657 ) ) ;
#3382=CARTESIAN_POINT ( 'NONE',  ( 36.60358173371529489, -284.6237833571632905, -234.7871824221999191 ) ) ;
#3383=CARTESIAN_POINT ( 'NONE',  ( -54.10599870879289597, -276.4591646791535595, -345.4030915490043867 ) ) ;
#3384=CARTESIAN_POINT ( 'NONE',  ( -91.04928535344082263, -288.1990336665144241, -324.4902966406356768 ) ) ;
#3385=CARTESIAN_POINT ( 'NONE',  ( -70.30981510752965846, -287.1296922317927738, -204.4394443781715722 ) ) ;
#3386=CARTESIAN_POINT ( 'NONE',  ( 3.714587149990489667, -278.2513697288731578, -331.9432199836292057 ) ) ;
#3387=CARTESIAN_POINT ( 'NONE',  ( -68.27895474457298519, -287.0789885570061415, -200.4791708890046777 ) ) ;
#3388=CARTESIAN_POINT ( 'NONE',  ( 13.28499688721336724, -284.3442213100884146, -325.6959008563357543 ) ) ;
#3389=CARTESIAN_POINT ( 'NONE',  ( -20.12403930961524168, -277.0036265471377988, -345.4661680429287571 ) ) ;
#3390=CARTESIAN_POINT ( 'NONE',  ( -106.3463232545784791, -277.9450047232013503, -304.6477661944054489 ) ) ;
#3391=CARTESIAN_POINT ( 'NONE',  ( -111.8245872750670031, -298.4574600745342536, -271.5092575864684932 ) ) ;
#3394=CARTESIAN_POINT ( 'NONE',  ( -37.23121733014565393, -296.1931139969674973, -194.5955937437999523 ) ) ;
#3396=CARTESIAN_POINT ( 'NONE',  ( -91.01731910912383228, -277.3478396063592868, -320.0020066101476459 ) ) ;
#3397=CARTESIAN_POINT ( 'NONE',  ( -68.69565184611099085, -274.8542161595667608, -200.4544609531145340 ) ) ;
#3398=CARTESIAN_POINT ( 'NONE',  ( 38.19189227883794047, -280.7835932419579876, -284.1270094048365422 ) ) ;
#3399=CARTESIAN_POINT ( 'NONE',  ( 35.56163497104553528, -289.1423880664242461, -257.3023228312590618 ) ) ;
#3400=CARTESIAN_POINT ( 'NONE',  ( -61.35485033385133846, -296.8784525281200786, -342.8461524688852933 ) ) ;
#3401=CARTESIAN_POINT ( 'NONE',  ( -47.56332316031804197, -296.3844183213226415, -346.2790153482373512 ) ) ;
#3402=CARTESIAN_POINT ( 'NONE',  ( 16.16908601960792780, -294.8132240842397778, -217.9741721522336206 ) ) ;
#3403=CARTESIAN_POINT ( 'NONE',  ( -8.518242664795220520, -278.4301388005070521, -201.3014573404978478 ) ) ;
#3404=CARTESIAN_POINT ( 'NONE',  ( 21.64223775218759371, -282.8452870759924167, -224.9288560693948398 ) ) ;
#3405=CARTESIAN_POINT ( 'NONE',  ( -35.06874290883403233, -296.1606666266059733, -195.9218606051179563 ) ) ;
#3406=CARTESIAN_POINT ( 'NONE',  ( -76.33086043225696926, -285.1640202527632368, -335.8920178884321217 ) ) ;
#3407=CARTESIAN_POINT ( 'NONE',  ( 29.70220634126613746, -286.8713741452664863, -300.1406900055482652 ) ) ;
#3408=CARTESIAN_POINT ( 'NONE',  ( -37.81643920958603644, -140.6726492126896346, -364.1437749989735835 ) ) ;
#3410=CARTESIAN_POINT ( 'NONE',  ( 34.77943607890461664, -287.3706479215621812, -281.8700862883184755 ) ) ;
#3412=CARTESIAN_POINT ( 'NONE',  ( -111.5722864269859116, -285.3890799960030904, -289.6826170217073013 ) ) ;
#3413=CARTESIAN_POINT ( 'NONE',  ( 31.28308989514621530, -276.2195874349703786, -295.4625486652283826 ) ) ;
#3414=CARTESIAN_POINT ( 'NONE',  ( 9.579703076757906999, -285.4765073871970458, -209.8103901689671318 ) ) ;
#3415=CARTESIAN_POINT ( 'NONE',  ( -97.21358883384220917, -290.1170594236804732, -222.4356607155498011 ) ) ;
#3416=CARTESIAN_POINT ( 'NONE',  ( 37.44553721366549581, -282.2755764260394926, -252.9918664540992097 ) ) ;
#3418=CARTESIAN_POINT ( 'NONE',  ( -56.40234970307031404, -281.3311188052444436, -196.4188603925978498 ) ) ;
#3419=CARTESIAN_POINT ( 'NONE',  ( 39.50835230792633723, -281.9516607562512149, -275.6552146410106729 ) ) ;
#3420=CARTESIAN_POINT ( 'NONE',  ( 17.40634833298269157, -278.4094976428775681, -226.7417163044926838 ) ) ;
#3423=CARTESIAN_POINT ( 'NONE',  ( 37.18202074190754303, -277.6398253042544297, -277.1613718337236492 ) ) ;
#3424=CARTESIAN_POINT ( 'NONE',  ( -113.0202178868561447, -270.5102741164896543, -296.2292133334984783 ) ) ;
#3426=CARTESIAN_POINT ( 'NONE',  ( 20.11802656611209628, -278.9112657782015958, -222.6943762391129553 ) ) ;
#3427=CARTESIAN_POINT ( 'NONE',  ( -69.29461257921681749, -296.9688094375072751, -204.6123229025582759 ) ) ;
#3428=CARTESIAN_POINT ( 'NONE',  ( -95.61020414936773193, -290.7389932783574977, -220.0984873618251640 ) ) ;
#3429=CARTESIAN_POINT ( 'NONE',  ( -97.39219751932952818, -246.9239084015011656, -331.4851807666400987 ) ) ;
#3431=CARTESIAN_POINT ( 'NONE',  ( -31.94293825058073466, -296.6932287952452612, -193.9516209903190997 ) ) ;
#3432=CARTESIAN_POINT ( 'NONE',  ( 16.57268045031483794, -285.2347499314938091, -219.9472256863061546 ) ) ;
#3433=CARTESIAN_POINT ( 'NONE',  ( 34.64963357485707718, -295.6476501391692864, -288.4750174734703592 ) ) ;
#3434=CARTESIAN_POINT ( 'NONE',  ( -5.600728758618639169, -287.7937102271188223, -204.0618423320328816 ) ) ;
#3436=CARTESIAN_POINT ( 'NONE',  ( 27.84619259727910290, -293.9603291448657956, -229.7223394935316492 ) ) ;
#3438=CARTESIAN_POINT ( 'NONE',  ( -98.16176580261897300, -285.6060052778029785, -229.8776886191627682 ) ) ;
#3439=CARTESIAN_POINT ( 'NONE',  ( -47.59369798343985281, -293.9746551386352849, -346.2749194801295971 ) ) ;
#3440=CARTESIAN_POINT ( 'NONE',  ( -98.02577560872533979, -290.7241780541166349, -317.4949890764902989 ) ) ;
#3441=CARTESIAN_POINT ( 'NONE',  ( -33.54867469438197958, -292.5910424320822472, -193.5162101395644640 ) ) ;
#3442=CARTESIAN_POINT ( 'NONE',  ( -72.35699666442870637, -289.6959892840354200, -334.4152280223494813 ) ) ;
#3445=CARTESIAN_POINT ( 'NONE',  ( 96.44228902283924754, -301.5705273522572156, -194.5544052147834577 ) ) ;
#3446=CARTESIAN_POINT ( 'NONE',  ( -87.76341052564968948, -272.1612075169296077, -212.6220725324359933 ) ) ;
#3447=CARTESIAN_POINT ( 'NONE',  ( 34.29786879288168677, -280.4102106372642993, -255.0966938950409144 ) ) ;
#3451=CARTESIAN_POINT ( 'NONE',  ( -1.324746964779585534, -274.0245518955879334, -202.3735750925492027 ) ) ;
#3452=CARTESIAN_POINT ( 'NONE',  ( -110.0501149628585438, -294.8751095925890127, -282.3692054820198223 ) ) ;
#3453=CARTESIAN_POINT ( 'NONE',  ( -91.85913063617145724, -279.7002230644374094, -320.8215270186369708 ) ) ;
#3454=CARTESIAN_POINT ( 'NONE',  ( 27.73049027741052086, -273.2105888176850499, -234.5261222635036518 ) ) ;
#3455=CARTESIAN_POINT ( 'NONE',  ( -108.2231049134757939, -298.0080769763791864, -251.2612192934299173 ) ) ;
#3456=CARTESIAN_POINT ( 'NONE',  ( -110.1095834582196602, -297.5096961944851728, -279.6586303020674222 ) ) ;
#3457=CARTESIAN_POINT ( 'NONE',  ( -112.9831370309887717, -298.2686637528121310, -261.1516968279346997 ) ) ;
#3458=CARTESIAN_POINT ( 'NONE',  ( 28.52243080689648380, -273.0861252370503962, -233.6433321265610630 ) ) ;
#3459=CARTESIAN_POINT ( 'NONE',  ( 35.30919848983042897, -294.3162414422748725, -278.9142396800737629 ) ) ;
#3460=CARTESIAN_POINT ( 'NONE',  ( -36.17875722034020214, -290.6417042956522891, -196.7684997398745566 ) ) ;
#3461=FACE_OUTER_BOUND ( 'NONE', #37309, .T. ) ;
#3462=CARTESIAN_POINT ( 'NONE',  ( 37.22403684347696640, -275.8070578647080424, -251.4012188966840995 ) ) ;
#3463=CARTESIAN_POINT ( 'NONE',  ( -68.28450880347773477, -273.8007633457644943, -204.2297779361963990 ) ) ;
#3464=CARTESIAN_POINT ( 'NONE',  ( 33.06000806390615310, -283.8796350802811617, -297.2312926088651466 ) ) ;
#3466=CARTESIAN_POINT ( 'NONE',  ( -37.33124170232879635, -281.7368201097845031, -346.8809497115246359 ) ) ;
#3470=CARTESIAN_POINT ( 'NONE',  ( -104.2651214110867102, -283.3523776848874149, -299.9221972969260719 ) ) ;
#3471=CARTESIAN_POINT ( 'NONE',  ( -70.94262198748015180, -281.4943253504089284, -337.5995480718307249 ) ) ;
#3473=CARTESIAN_POINT ( 'NONE',  ( 33.07497690071242857, -274.4081549606615908, -291.7791999513033261 ) ) ;
#3474=CARTESIAN_POINT ( 'NONE',  ( -23.79561910030680849, -282.2252611632882804, -196.5423384039622192 ) ) ;
#3477=CARTESIAN_POINT ( 'NONE',  ( -87.49435193961841151, -271.7662184468114219, -212.9224195425988171 ) ) ;
#3478=CARTESIAN_POINT ( 'NONE',  ( -110.6897125428610025, -280.3417573901916739, -286.7957614591096558 ) ) ;
#3480=CARTESIAN_POINT ( 'NONE',  ( -106.6158994474202757, -286.8657778370662186, -240.0573691442952793 ) ) ;
#3482=CARTESIAN_POINT ( 'NONE',  ( -110.7266578267132502, -288.7515249627732601, -254.8199309094176783 ) ) ;
#3484=CARTESIAN_POINT ( 'NONE',  ( -98.77153666896752782, -295.9018593688907686, -230.1007066985058316 ) ) ;
#3485=CARTESIAN_POINT ( 'NONE',  ( -71.76624294165712570, -287.6516547220033999, -336.1464198544258579 ) ) ;
#3486=CARTESIAN_POINT ( 'NONE',  ( 121.1498776811041438, 150.0802918209077177, -263.8330885344481658 ) ) ;
#3487=CARTESIAN_POINT ( 'NONE',  ( -107.6726829452816219, -294.8918204399934098, -244.1623968445080095 ) ) ;
#3488=CARTESIAN_POINT ( 'NONE',  ( 1.188457573889697860, -285.0366859289206900, -204.4813979563307385 ) ) ;
#3489=CARTESIAN_POINT ( 'NONE',  ( 35.27625943179678103, -283.3248736587961503, -283.5877328220953473 ) ) ;
#3490=CARTESIAN_POINT ( 'NONE',  ( 3.975652429553107048, -280.7441613301439247, -334.1951580907712582 ) ) ;
#3491=CARTESIAN_POINT ( 'NONE',  ( -37.26801856798356027, -289.0512044463033021, -343.3610807978087678 ) ) ;
#3493=CARTESIAN_POINT ( 'NONE',  ( 19.82113896954361465, -283.6280743775568567, -316.7251846059284617 ) ) ;
#3494=CARTESIAN_POINT ( 'NONE',  ( 19.79572939634006090, -281.7108435265626554, -224.6673998703409154 ) ) ;
#3495=CARTESIAN_POINT ( 'NONE',  ( 37.96200453370386896, -289.5825242995225040, -274.3110319910481962 ) ) ;
#3497=CARTESIAN_POINT ( 'NONE',  ( -82.97228390446436208, -297.6139512576797301, -208.2718905325717174 ) ) ;
#3500=CARTESIAN_POINT ( 'NONE',  ( -81.25038677240452500, -273.4736917697527474, -207.0428328662378306 ) ) ;
#3501=CARTESIAN_POINT ( 'NONE',  ( -4.123262171867538406, -294.4721556704471368, -203.5009228801643530 ) ) ;
#3503=CARTESIAN_POINT ( 'NONE',  ( -95.95921662488163406, -286.4090924074130839, -317.1477375740089997 ) ) ;
#3505=CARTESIAN_POINT ( 'NONE',  ( 37.79886013720064142, -273.5266078969362411, -268.3800509541516703 ) ) ;
#3507=CARTESIAN_POINT ( 'NONE',  ( -112.8626095561200771, -294.8188545096006692, -280.8988274138584416 ) ) ;
#3508=CARTESIAN_POINT ( 'NONE',  ( -62.05636646272959922, -273.0707073773173192, -201.5637493112703282 ) ) ;
#3509=AXIS2_PLACEMENT_3D ( 'NONE', #17354, #44350, #80806 ) ;
#3510=CARTESIAN_POINT ( 'NONE',  ( -91.27973232351980926, -292.7876233583033354, -220.1289463421949790 ) ) ;
#3511=CARTESIAN_POINT ( 'NONE',  ( -59.22667057881314179, -285.0993336956092890, -341.1187548907683436 ) ) ;
#3512=CARTESIAN_POINT ( 'NONE',  ( -112.2864870736867289, -291.7888547884392665, -285.3231724539863876 ) ) ;
#3513=CARTESIAN_POINT ( 'NONE',  ( -104.1872876013020885, -292.3528703765999808, -233.1459905883267822 ) ) ;
#3514=CARTESIAN_POINT ( 'NONE',  ( 28.39362824236933491, -293.8165028841322624, -302.2246007315227416 ) ) ;
#3515=CARTESIAN_POINT ( 'NONE',  ( 7.048319744136891885, -290.4483194718962409, -330.8785390666133139 ) ) ;
#3516=CARTESIAN_POINT ( 'NONE',  ( 22.87398460134540557, -281.0760973511481211, -222.3498315182758631 ) ) ;
#3517=CARTESIAN_POINT ( 'NONE',  ( -112.3424223613341724, -294.7489488954487911, -261.1847427880285295 ) ) ;
#3518=CARTESIAN_POINT ( 'NONE',  ( -27.37420368595265430, -282.7622862379806179, -346.7666173154133276 ) ) ;
#3520=CARTESIAN_POINT ( 'NONE',  ( 28.22328208483245149, -278.0096016008662900, -306.1494825789188212 ) ) ;
#3521=CARTESIAN_POINT ( 'NONE',  ( -9.685128554203979334, -274.8342426744605973, -340.8977717842163315 ) ) ;
#3523=CARTESIAN_POINT ( 'NONE',  ( -92.60978701811066571, -283.3793437537340765, -318.1653762170193431 ) ) ;
#3525=CARTESIAN_POINT ( 'NONE',  ( -48.07838628637967560, -281.1236714209066463, -194.4607814239770107 ) ) ;
#3526=CARTESIAN_POINT ( 'NONE',  ( 1.413272689442203855, -285.6154625031711021, -204.0821678239133803 ) ) ;
#3527=CARTESIAN_POINT ( 'NONE',  ( 9.472692893479200293, -294.4657847708367058, -212.9676436195597091 ) ) ;
#3528=CARTESIAN_POINT ( 'NONE',  ( 38.82475190748067462, -277.1980820771216258, -273.9853798329471601 ) ) ;
#3529=CARTESIAN_POINT ( 'NONE',  ( 27.24158974425489887, -277.4094432712955722, -311.4754408556286194 ) ) ;
#3530=CARTESIAN_POINT ( 'NONE',  ( -110.1685116794591721, -278.3100721470262329, -276.0767695804867117 ) ) ;
#3531=CARTESIAN_POINT ( 'NONE',  ( -109.5372873558532802, -274.7792576125245319, -251.1983830590123148 ) ) ;
#3532=CARTESIAN_POINT ( 'NONE',  ( -10.05841032550461733, -284.4089916781757097, -200.6647522803869492 ) ) ;
#3533=CARTESIAN_POINT ( 'NONE',  ( 32.20909583356594652, -293.6431795383152803, -303.4767414905147689 ) ) ;
#3534=CARTESIAN_POINT ( 'NONE',  ( -86.84904272021957183, -291.3273215102551035, -328.3567692955385837 ) ) ;
#3536=CARTESIAN_POINT ( 'NONE',  ( 29.02417964233303849, -292.0521722741974600, -239.0997151428993845 ) ) ;
#3538=CARTESIAN_POINT ( 'NONE',  ( -86.12280831207357323, -289.9660489227205744, -211.4790834090941303 ) ) ;
#3539=CARTESIAN_POINT ( 'NONE',  ( 2.255529487390719012, -292.2650364333858874, -208.9485746055341622 ) ) ;
#3540=VERTEX_POINT ( 'NONE', #91205 ) ;
#3541=CARTESIAN_POINT ( 'NONE',  ( -95.21596241793501747, -290.9488912308358408, -320.6807192806642206 ) ) ;
#3542=CARTESIAN_POINT ( 'NONE',  ( -110.0684122584599862, -279.3074120160384837, -262.4782581799385071 ) ) ;
#3544=CARTESIAN_POINT ( 'NONE',  ( -98.83631042565870928, -296.0846984200247789, -224.5144804261545062 ) ) ;
#3545=CARTESIAN_POINT ( 'NONE',  ( -52.16177603630362114, -286.5187603413301076, -194.8503335397373917 ) ) ;
#3546=CARTESIAN_POINT ( 'NONE',  ( 27.11773386100906080, -287.3324524171187591, -228.2811267598260088 ) ) ;
#3547=CARTESIAN_POINT ( 'NONE',  ( -97.37574256147604501, -285.4646735099198054, -228.7697798428477540 ) ) ;
#3548=CARTESIAN_POINT ( 'NONE',  ( -31.54385115895311387, -124.1296239072845680, -364.1778657101864383 ) ) ;
#3549=CARTESIAN_POINT ( 'NONE',  ( -110.5300065284289133, -264.7307192410654579, -306.1878980822340850 ) ) ;
#3550=CARTESIAN_POINT ( 'NONE',  ( -31.03177537408224751, -124.7070154724701752, -360.4556306706562623 ) ) ;
#3551=CARTESIAN_POINT ( 'NONE',  ( -94.58576116420519497, -277.1071319848362009, -315.9411938318368698 ) ) ;
#3552=CARTESIAN_POINT ( 'NONE',  ( 21.07494522676942950, -275.0922978967715267, -314.6524446726106135 ) ) ;
#3553=CARTESIAN_POINT ( 'NONE',  ( -60.12388022359375128, -297.2723495997484520, -196.8175532766127276 ) ) ;
#3554=CARTESIAN_POINT ( 'NONE',  ( -97.02394130038283038, -247.4898175441587114, -331.8706397708260738 ) ) ;
#3555=CARTESIAN_POINT ( 'NONE',  ( -84.57516265379381082, -276.3718005307977137, -330.6139778956907094 ) ) ;
#3556=CARTESIAN_POINT ( 'NONE',  ( -38.11513081123835889, -275.8024718723389697, -196.3518224758765314 ) ) ;
#3557=CARTESIAN_POINT ( 'NONE',  ( -105.1678373823866508, -290.6796861829718637, -297.6557278294694129 ) ) ;
#3558=CARTESIAN_POINT ( 'NONE',  ( -111.4690222184587043, -297.6111311020603694, -249.9332731992617767 ) ) ;
#3559=CARTESIAN_POINT ( 'NONE',  ( -89.57113311769904840, -297.8319755070070300, -213.7945775454860495 ) ) ;
#3560=CARTESIAN_POINT ( 'NONE',  ( 17.97381884032833099, -294.3974273772245169, -318.0162292550816119 ) ) ;
#3563=CARTESIAN_POINT ( 'NONE',  ( -56.53420651391186169, -279.2176532685523398, -343.4970207104573205 ) ) ;
#3564=CARTESIAN_POINT ( 'NONE',  ( -30.22682948699986483, -282.4720686814482633, -346.9699002399244137 ) ) ;
#3566=CARTESIAN_POINT ( 'NONE',  ( -40.50396707637281679, -278.0341096356804087, -343.5406132354212332 ) ) ;
#3567=CARTESIAN_POINT ( 'NONE',  ( 36.26284111494198470, -277.5516729311813720, -289.2382344107984977 ) ) ;
#3568=CARTESIAN_POINT ( 'NONE',  ( -60.68575216430463826, -296.3181406805940128, -200.5187549589553839 ) ) ;
#3570=CARTESIAN_POINT ( 'NONE',  ( -78.63025341943485103, -277.7918684300138352, -330.6244583185356873 ) ) ;
#3572=CARTESIAN_POINT ( 'NONE',  ( -90.05952426016648360, -274.1329562602711007, -214.3868399119125456 ) ) ;
#3573=CARTESIAN_POINT ( 'NONE',  ( 38.59892950167494519, -286.3592783143711245, -280.0772776289361445 ) ) ;
#3574=CARTESIAN_POINT ( 'NONE',  ( -46.65846988999888367, -275.9340286228207333, -195.9420448328806401 ) ) ;
#3575=CARTESIAN_POINT ( 'NONE',  ( 38.96705684354925125, -274.0655611780182994, -265.4955255711364543 ) ) ;
#3578=CARTESIAN_POINT ( 'NONE',  ( -10.67475059123048631, -287.8925288928151076, -338.5438257208471100 ) ) ;
#3580=CARTESIAN_POINT ( 'NONE',  ( -110.5909832594162765, -283.6055915651521104, -293.8108658896078964 ) ) ;
#3581=CARTESIAN_POINT ( 'NONE',  ( 35.70002379452798635, -279.9475316401529312, -282.3143845139392170 ) ) ;
#3582=CARTESIAN_POINT ( 'NONE',  ( 35.72256530037758893, -280.2471157571049503, -279.5496743247740028 ) ) ;
#3583=CARTESIAN_POINT ( 'NONE',  ( -74.24874123376558543, -283.6373982981772883, -205.6997258425355426 ) ) ;
#3584=CARTESIAN_POINT ( 'NONE',  ( 29.42458971303385340, -290.0054700535752659, -304.6389638658780541 ) ) ;
#3585=CARTESIAN_POINT ( 'NONE',  ( -103.7355515119771781, -280.1791238356550480, -238.9528368796921995 ) ) ;
#3587=CARTESIAN_POINT ( 'NONE',  ( 27.18488080863017231, -279.4146534923528407, -229.7312065776307293 ) ) ;
#3588=CARTESIAN_POINT ( 'NONE',  ( 5.336681734716932191, -294.6298804052118498, -208.6881387458344363 ) ) ;
#3590=CARTESIAN_POINT ( 'NONE',  ( -90.33519128877667015, -277.5549640475629189, -215.8298763579868478 ) ) ;
#3591=CARTESIAN_POINT ( 'NONE',  ( -43.20700921346766421, -277.7795873713844230, -343.2273709229162364 ) ) ;
#3592=CARTESIAN_POINT ( 'NONE',  ( -41.44300898866784166, -285.1037115954483738, -345.4668974981497627 ) ) ;
#3594=CARTESIAN_POINT ( 'NONE',  ( -92.52410291393324826, -291.7542614080916223, -322.0525459733080993 ) ) ;
#3597=CARTESIAN_POINT ( 'NONE',  ( -4.832952116147695598, -285.6666530723716733, -200.7382760127721895 ) ) ;
#3598=CARTESIAN_POINT ( 'NONE',  ( -79.97644140347784969, -289.8648009274541550, -210.0596393592840911 ) ) ;
#3600=CARTESIAN_POINT ( 'NONE',  ( 35.11465735488442874, -274.0748087476350179, -257.9850623104874217 ) ) ;
#3601=CARTESIAN_POINT ( 'NONE',  ( -3.799391091954892552, -292.7444360309395393, -336.6005652980742866 ) ) ;
#3604=CARTESIAN_POINT ( 'NONE',  ( -14.05941338440898036, -290.8285501941077200, -197.6376102078408792 ) ) ;
#3605=CARTESIAN_POINT ( 'NONE',  ( -110.8914037317769896, -286.0730426712937060, -276.4341331833798563 ) ) ;
#3606=CARTESIAN_POINT ( 'NONE',  ( -75.17880751458058342, -287.7890861640981939, -336.2574556549772637 ) ) ;
#3607=CARTESIAN_POINT ( 'NONE',  ( -38.65346954131330648, -287.4606941471247410, -196.7709972478338329 ) ) ;
#3610=CARTESIAN_POINT ( 'NONE',  ( 22.09884203058636132, -288.9499373939734710, -313.0158208316170203 ) ) ;
#3611=CARTESIAN_POINT ( 'NONE',  ( 34.70681222247446129, -295.2487667415485930, -248.2835576237800126 ) ) ;
#3612=CARTESIAN_POINT ( 'NONE',  ( -100.8992325856211068, -276.0845769087823101, -311.3192643314317252 ) ) ;
#3613=CARTESIAN_POINT ( 'NONE',  ( -67.69636223418849852, -277.7730056753987924, -341.1024692560662857 ) ) ;
#3614=CARTESIAN_POINT ( 'NONE',  ( 26.84233109548847906, -291.0993841984039818, -230.3908562936944122 ) ) ;
#3615=CARTESIAN_POINT ( 'NONE',  ( -113.7662432301547710, -278.4293597551597941, -280.1794997208239124 ) ) ;
#3616=CARTESIAN_POINT ( 'NONE',  ( -96.61009421258725638, -299.1565390367795771, -224.9629286694865016 ) ) ;
#3618=CARTESIAN_POINT ( 'NONE',  ( -110.3786324335668922, -282.3324557148184795, -287.4645182672546753 ) ) ;
#3620=CARTESIAN_POINT ( 'NONE',  ( -109.6954169800915366, -276.4755713682384908, -287.0249116973764671 ) ) ;
#3621=CARTESIAN_POINT ( 'NONE',  ( 36.88807596914821829, -279.6896477438029933, -281.0821715460117503 ) ) ;
#3623=CARTESIAN_POINT ( 'NONE',  ( 19.34901374047956324, -274.7318770703203654, -321.4577720552351821 ) ) ;
#3624=CARTESIAN_POINT ( 'NONE',  ( -110.4264030661165066, -298.2008373491525504, -260.5231914145043675 ) ) ;
#3625=CARTESIAN_POINT ( 'NONE',  ( -76.61147981202276469, -282.4846526728620688, -336.2966422407261575 ) ) ;
#3626=CARTESIAN_POINT ( 'NONE',  ( -70.58503270139516417, -298.5438992151777029, -205.0915916167130320 ) ) ;
#3627=CARTESIAN_POINT ( 'NONE',  ( -110.3476246162948797, -298.1586358163755222, -247.3067130482227185 ) ) ;
#3628=CARTESIAN_POINT ( 'NONE',  ( 5.192506653319919785, -274.3117287078989079, -210.9443556489674165 ) ) ;
#3629=CARTESIAN_POINT ( 'NONE',  ( 3.303550686920755375, -294.5981021510733058, -207.2681548189215448 ) ) ;
#3630=CARTESIAN_POINT ( 'NONE',  ( 27.13659901274048281, -287.1658781473803970, -228.2713455383054679 ) ) ;
#3631=CARTESIAN_POINT ( 'NONE',  ( -3.301641916264301813, -274.7471367666977926, -338.0629276371942069 ) ) ;
#3632=CARTESIAN_POINT ( 'NONE',  ( 25.85049158197741548, -287.9679283919724639, -314.4497864515938090 ) ) ;
#3633=CARTESIAN_POINT ( 'NONE',  ( 23.73690771995800119, -286.0509875304440470, -229.8612124768762328 ) ) ;
#3634=CARTESIAN_POINT ( 'NONE',  ( -108.5244133883725652, -288.8591520860207993, -246.5762767011976564 ) ) ;
#3636=CARTESIAN_POINT ( 'NONE',  ( 206.6943913402143096, 294.1769577359763161, -83.83314285352493300 ) ) ;
#3638=CARTESIAN_POINT ( 'NONE',  ( -3.343318345540888803, -288.0984722136330447, -335.0862926492917495 ) ) ;
#3640=CARTESIAN_POINT ( 'NONE',  ( -97.85153049825210303, -284.8602827561805384, -317.5986098996201008 ) ) ;
#3641=CARTESIAN_POINT ( 'NONE',  ( 10.98000521840325838, -291.7606223035207904, -210.6451465341437483 ) ) ;
#3642=CARTESIAN_POINT ( 'NONE',  ( 35.40583081042965574, -282.8643995261323312, -247.6843201971592805 ) ) ;
#3643=CARTESIAN_POINT ( 'NONE',  ( -3.888463415681657320, -281.7993682370669717, -201.5413225496155576 ) ) ;
#3644=CARTESIAN_POINT ( 'NONE',  ( -92.56052022569977566, -283.7049582715205815, -318.1282502806257071 ) ) ;
#3645=CARTESIAN_POINT ( 'NONE',  ( 18.02432890966275636, -278.2588308072120640, -320.9728043955709040 ) ) ;
#3646=CARTESIAN_POINT ( 'NONE',  ( -54.59516618233048746, -297.8363351003297339, -195.3190104087792918 ) ) ;
#3648=CARTESIAN_POINT ( 'NONE',  ( -81.37981066230648253, -274.7545378001894960, -211.4594357926004307 ) ) ;
#3649=CARTESIAN_POINT ( 'NONE',  ( 0.7700471852684900309, -290.5832673472678493, -206.1790214181901320 ) ) ;
#3650=CARTESIAN_POINT ( 'NONE',  ( -37.81075464249324369, -296.9664671818636066, -197.0535054000108346 ) ) ;
#3653=CARTESIAN_POINT ( 'NONE',  ( -108.7668310379991397, -286.1996917792465638, -291.3771489139386404 ) ) ;
#3655=CARTESIAN_POINT ( 'NONE',  ( -32.02017785781833936, -296.0661944938649413, -346.8803577203190684 ) ) ;
#3657=CARTESIAN_POINT ( 'NONE',  ( -109.0779264960525126, -285.0182938389965557, -284.4254876788514252 ) ) ;
#3658=CARTESIAN_POINT ( 'NONE',  ( 27.44379568282640136, -275.1533809843029417, -311.6382920504752292 ) ) ;
#3659=CARTESIAN_POINT ( 'NONE',  ( 20.29678017065466733, -293.5131461247013931, -219.4381975904448723 ) ) ;
#3660=CARTESIAN_POINT ( 'NONE',  ( 30.32935644297891642, -285.2461718969747722, -236.2886425755122559 ) ) ;
#3661=CARTESIAN_POINT ( 'NONE',  ( 4.126568248832680474, -292.9275303271610369, -205.4432764109110394 ) ) ;
#3662=CARTESIAN_POINT ( 'NONE',  ( -96.57328127619301483, -290.2883733847293684, -313.0660039034881947 ) ) ;
#3666=CARTESIAN_POINT ( 'NONE',  ( -62.22388460320987491, -183.0710032457758984, -358.7722912303554494 ) ) ;
#3667=CARTESIAN_POINT ( 'NONE',  ( -57.59075369304125758, -287.3156083290446077, -196.7353183839019550 ) ) ;
#3668=CARTESIAN_POINT ( 'NONE',  ( -95.95921662488163406, -294.6952119285919025, -223.5744983911110353 ) ) ;
#3671=CARTESIAN_POINT ( 'NONE',  ( 16.04156061211757489, -281.1934707343594937, -320.6782800191246565 ) ) ;
#3672=CARTESIAN_POINT ( 'NONE',  ( -112.9746097129493592, -278.3990453635024096, -255.9586054810243922 ) ) ;
#3673=CARTESIAN_POINT ( 'NONE',  ( -13.75458084390644231, -282.3590026451987569, -199.2874991544501313 ) ) ;
#3674=CARTESIAN_POINT ( 'NONE',  ( -68.72028664152445288, -197.1574858626671300, -358.6428543488109426 ) ) ;
#3676=CARTESIAN_POINT ( 'NONE',  ( 22.92688668245770245, -280.7594868724583534, -317.3535635459220998 ) ) ;
#3677=CARTESIAN_POINT ( 'NONE',  ( 14.29518050955971908, -284.8017966785216117, -216.3872835249163415 ) ) ;
#3678=CARTESIAN_POINT ( 'NONE',  ( -108.9424241297686535, -274.7299519248360866, -245.5893234993298506 ) ) ;
#3680=CARTESIAN_POINT ( 'NONE',  ( -6.733421242427103159, -295.1314706440206805, -336.7020684243057076 ) ) ;
#3682=CARTESIAN_POINT ( 'NONE',  ( 0.1750993051216313823, -291.2478782896370717, -207.1651272999152980 ) ) ;
#3683=CARTESIAN_POINT ( 'NONE',  ( 22.56681797367697584, -276.8507392544338472, -318.5927596699377773 ) ) ;
#3684=CARTESIAN_POINT ( 'NONE',  ( -54.21153688493372869, -273.8293901800537924, -199.3371177587120542 ) ) ;
#3685=CARTESIAN_POINT ( 'NONE',  ( 39.01095305913688804, -274.3753454015922557, -262.6252497561658288 ) ) ;
#3687=CARTESIAN_POINT ( 'NONE',  ( -82.69117329601709798, -271.4326210128701291, -210.5603382261614058 ) ) ;
#3688=CARTESIAN_POINT ( 'NONE',  ( -64.04315138647687888, -296.8190070920826429, -341.9546846855083118 ) ) ;
#3691=CARTESIAN_POINT ( 'NONE',  ( -99.28489239726592075, -285.0911461414118548, -309.6641206029707405 ) ) ;
#3692=CARTESIAN_POINT ( 'NONE',  ( 36.88063014320469080, -283.5193611751342360, -286.7007127241964213 ) ) ;
#3693=CARTESIAN_POINT ( 'NONE',  ( -109.5204537167712289, -284.0543398857845432, -258.7008559994420125 ) ) ;
#3694=CARTESIAN_POINT ( 'NONE',  ( -35.11367763140418674, -275.4235795490523060, -344.1274811344654267 ) ) ;
#3695=CARTESIAN_POINT ( 'NONE',  ( -15.75100204404952109, -284.6302552625655835, -341.3872204692429477 ) ) ;
#3696=CARTESIAN_POINT ( 'NONE',  ( -110.5954289105286250, -276.9210866731372107, -278.8506460073057838 ) ) ;
#3697=CARTESIAN_POINT ( 'NONE',  ( 34.67459842992152375, -276.4517726080438820, -256.6542286077366271 ) ) ;
#3699=CARTESIAN_POINT ( 'NONE',  ( -28.25426863066250505, -280.9673716393867835, -194.0083440244762301 ) ) ;
#3703=CARTESIAN_POINT ( 'NONE',  ( -102.9823526865151138, -286.9136298341684324, -232.4201070035155396 ) ) ;
#3704=CARTESIAN_POINT ( 'NONE',  ( -73.39085345530745030, -294.7406820238770138, -334.0247675129881486 ) ) ;
#3705=CARTESIAN_POINT ( 'NONE',  ( -112.2161213889790474, -290.1202169613839601, -252.8358839466416441 ) ) ;
#3706=CARTESIAN_POINT ( 'NONE',  ( 29.12812112663493025, -286.2269449983073173, -302.9147179869371485 ) ) ;
#3707=CARTESIAN_POINT ( 'NONE',  ( 15.46485560699442985, -285.3918276152409135, -219.1083854862778821 ) ) ;
#3708=CARTESIAN_POINT ( 'NONE',  ( -75.48285505297796760, -289.7761964459410251, -206.8723858681778438 ) ) ;
#3709=CARTESIAN_POINT ( 'NONE',  ( -109.3661999113004981, -285.5718668317051652, -284.4891729368653728 ) ) ;
#3710=CARTESIAN_POINT ( 'NONE',  ( 27.35743948046766505, -274.0589582028262612, -308.2955611787468229 ) ) ;
#3711=CARTESIAN_POINT ( 'NONE',  ( 22.64493826663130349, -286.5869506597848044, -317.3719459951165049 ) ) ;
#3712=CARTESIAN_POINT ( 'NONE',  ( -54.53160599625301330, -287.8314300863208359, -197.3576401074107025 ) ) ;
#3713=CARTESIAN_POINT ( 'NONE',  ( 25.88847412566088479, -286.0993400144516272, -311.1015168225341085 ) ) ;
#3714=CARTESIAN_POINT ( 'NONE',  ( 18.68207087875009620, -283.1614534672724517, -317.5477972199113310 ) ) ;
#3715=CARTESIAN_POINT ( 'NONE',  ( 17.32929186436410163, -290.2739087983973718, -321.9470759671938254 ) ) ;
#3718=CARTESIAN_POINT ( 'NONE',  ( -87.62850582987663017, -297.6675395369700823, -326.8276375493790624 ) ) ;
#3719=CARTESIAN_POINT ( 'NONE',  ( -19.02203114442400178, -278.2876494383350519, -197.5791950613629240 ) ) ;
#3720=CARTESIAN_POINT ( 'NONE',  ( -22.21554921374996283, -291.4381808060925891, -194.9719300890212708 ) ) ;
#3721=CARTESIAN_POINT ( 'NONE',  ( -110.0607041098306240, -295.1162397386514158, -257.7759331969653545 ) ) ;
#3722=CARTESIAN_POINT ( 'NONE',  ( 21.73531356265890579, -279.6279216616588315, -226.6232302346700749 ) ) ;
#3723=CARTESIAN_POINT ( 'NONE',  ( 0.2006842507856418378, -272.6359761036351301, -206.0665076447548643 ) ) ;
#3724=CARTESIAN_POINT ( 'NONE',  ( -75.90264450403937246, -296.8936097310100308, -332.9847849940167634 ) ) ;
#3726=CARTESIAN_POINT ( 'NONE',  ( -99.08015730504273222, -271.7300684382305462, -225.2515336869703049 ) ) ;
#3727=CARTESIAN_POINT ( 'NONE',  ( 37.60307598746469893, -291.9519350583364599, -282.9799375716426084 ) ) ;
#3728=VECTOR ( 'NONE', #17944, 999.9999999999998863 ) ;
#3729=CARTESIAN_POINT ( 'NONE',  ( -30.77230205459084900, -293.5620974422297422, -197.0657025320491016 ) ) ;
#3731=CARTESIAN_POINT ( 'NONE',  ( 14.98386275671792589, -293.6160892113402952, -219.1550446047386060 ) ) ;
#3733=CARTESIAN_POINT ( 'NONE',  ( -27.61004275948390685, -280.9493661771480220, -345.1375085902362798 ) ) ;
#3734=CARTESIAN_POINT ( 'NONE',  ( 20.52320543901548433, -294.1787170949178858, -314.8861090188129879 ) ) ;
#3735=CARTESIAN_POINT ( 'NONE',  ( 32.39238987560119654, -281.9716586663358271, -303.1387913265050429 ) ) ;
#3736=CARTESIAN_POINT ( 'NONE',  ( -106.9883179038249779, -283.7987696096448644, -303.1497276486421697 ) ) ;
#3737=CARTESIAN_POINT ( 'NONE',  ( -99.81640266325914013, -289.1104353168295233, -229.0731080423128105 ) ) ;
#3739=CARTESIAN_POINT ( 'NONE',  ( 22.84401450027144875, -280.6646525542469135, -317.2905150132684753 ) ) ;
#3740=CIRCLE ( 'NONE', #6802, 2.939656322713313230 ) ;
#3742=CARTESIAN_POINT ( 'NONE',  ( -7.054705697281143273, -287.5843340915924955, -340.8323111664559519 ) ) ;
#3744=CARTESIAN_POINT ( 'NONE',  ( -76.06061488172476004, -297.1785181648194225, -333.2481186419474852 ) ) ;
#3745=CARTESIAN_POINT ( 'NONE',  ( 21.29025772054045973, -277.6418650265628685, -319.3600956610622461 ) ) ;
#3746=CARTESIAN_POINT ( 'NONE',  ( -51.82740420475825260, -279.5285163502910564, -198.7394640599044067 ) ) ;
#3747=CARTESIAN_POINT ( 'NONE',  ( 23.97394127447170931, -293.0979133398607246, -223.7626877676976846 ) ) ;
#3748=CARTESIAN_POINT ( 'NONE',  ( -105.7132288800199262, -282.2121521082460163, -302.5270666125585990 ) ) ;
#3749=CARTESIAN_POINT ( 'NONE',  ( -68.16940249262060547, -279.4571092204822094, -338.7465830200557093 ) ) ;
#3750=CARTESIAN_POINT ( 'NONE',  ( 32.85805851504282771, -292.3335562041454523, -249.3199720749372261 ) ) ;
#3751=CARTESIAN_POINT ( 'NONE',  ( -77.11957347515530614, -295.5188283455943292, -206.7787191624978504 ) ) ;
#3754=CARTESIAN_POINT ( 'NONE',  ( -23.51332835650195108, -294.3783842667656927, -342.1537197203543315 ) ) ;
#3756=CARTESIAN_POINT ( 'NONE',  ( -82.08285599513421005, -288.9094976428775681, -214.2051214447836571 ) ) ;
#3757=CARTESIAN_POINT ( 'NONE',  ( -37.59482026529267529, -297.1078084665533652, -193.5968284698001298 ) ) ;
#3758=CARTESIAN_POINT ( 'NONE',  ( -69.60026389723520879, -286.9515539124382713, -200.9733374609629379 ) ) ;
#3759=CARTESIAN_POINT ( 'NONE',  ( -61.25701600895228438, -289.2048696744967060, -339.3325444634945711 ) ) ;
#3760=CARTESIAN_POINT ( 'NONE',  ( -110.3111115768619470, -280.2115630193436004, -259.7023745579906517 ) ) ;
#3761=CARTESIAN_POINT ( 'NONE',  ( -58.21168634846085865, -299.5388727493933061, -199.3511349760614735 ) ) ;
#3762=CARTESIAN_POINT ( 'NONE',  ( -54.05920378112192992, -276.0663880267032937, -341.8814087185648987 ) ) ;
#3764=CARTESIAN_POINT ( 'NONE',  ( -23.36033430842553571, -297.8894392957309947, -193.3830261749414774 ) ) ;
#3765=CARTESIAN_POINT ( 'NONE',  ( -87.68560857433259059, -291.6815103985820201, -325.2653652623214384 ) ) ;
#3766=CARTESIAN_POINT ( 'NONE',  ( 38.44370002599556102, -295.2587489999416448, -278.7859613990530647 ) ) ;
#3767=CARTESIAN_POINT ( 'NONE',  ( -112.5627052039163516, -274.5519900738179331, -270.3865807095182276 ) ) ;
#3768=CARTESIAN_POINT ( 'NONE',  ( -95.02588653217055992, -290.5715431880959159, -315.2859854738908325 ) ) ;
#3770=CARTESIAN_POINT ( 'NONE',  ( 19.46847308635654983, -291.0017227332807579, -220.2125791070446894 ) ) ;
#3771=CARTESIAN_POINT ( 'NONE',  ( -9.124202496769562742, -298.7296733842057392, -193.3807113113939522 ) ) ;
#3772=CARTESIAN_POINT ( 'NONE',  ( -79.73687535343847799, -297.1277458130988975, -210.9074670912553984 ) ) ;
#3775=CARTESIAN_POINT ( 'NONE',  ( -112.4925842252274890, -292.2392415583480556, -257.1303820601103212 ) ) ;
#3776=CARTESIAN_POINT ( 'NONE',  ( -99.86837403722181250, -292.4090924074130839, -320.2651865833026363 ) ) ;
#3778=CARTESIAN_POINT ( 'NONE',  ( -109.5229372111426045, -286.2972642340722018, -290.1552565137893680 ) ) ;
#3780=CARTESIAN_POINT ( 'NONE',  ( -40.83566927194004847, -272.0080689501005509, -195.5584416224066615 ) ) ;
#3781=CARTESIAN_POINT ( 'NONE',  ( -86.27480106415140426, -275.2875578507015462, -214.1954637909017549 ) ) ;
#3782=CARTESIAN_POINT ( 'NONE',  ( 31.19085896907123612, -291.2478215303064530, -241.1670925712065809 ) ) ;
#3783=CARTESIAN_POINT ( 'NONE',  ( -111.8465745835718366, -280.2367701674981504, -284.1919722268178816 ) ) ;
#3785=CARTESIAN_POINT ( 'NONE',  ( -48.35221062882412468, -282.5445874753498856, -342.6291007028255535 ) ) ;
#3786=CARTESIAN_POINT ( 'NONE',  ( -111.0440035944138231, -279.8986946984858264, -249.1605761525999299 ) ) ;
#3787=CARTESIAN_POINT ( 'NONE',  ( 23.44165430925463767, -279.7217804362036873, -223.7200259240646574 ) ) ;
#3789=CARTESIAN_POINT ( 'NONE',  ( 83.10068444444905822, 82.68374727650824241, -299.4140318971746524 ) ) ;
#3790=CARTESIAN_POINT ( 'NONE',  ( 26.72756007566194825, -275.9356431648753869, -228.0769588946166380 ) ) ;
#3792=CARTESIAN_POINT ( 'NONE',  ( -49.62686765597128868, -275.4184753970764632, -194.9965585817814713 ) ) ;
#3793=CARTESIAN_POINT ( 'NONE',  ( 7.450504543161046378, -278.9090924074131408, -326.4764044574609443 ) ) ;
#3796=B_SPLINE_CURVE_WITH_KNOTS ( 'NONE', 3,
 ( #44129, #45509, #60232, #80131, #23763, #53094, #38882, #73034, #8163, #67791 ),
 .UNSPECIFIED., .F., .F.,
 ( 4, 2, 2, 2, 4 ),
 ( 0.5000000000000000000, 0.5447723136181439330, 0.5895446272362879769, 0.6343169408544320209, 0.6790892544725759539 ),
 .UNSPECIFIED. ) ;
#3797=FACE_OUTER_BOUND ( 'NONE', #60628, .T. ) ;
#3798=CARTESIAN_POINT ( 'NONE',  ( -88.86860724608207818, -290.8767907922493237, -322.5071045599775061 ) ) ;
#3799=CARTESIAN_POINT ( 'NONE',  ( 21.29374681377383638, -288.6542313100443948, -222.0303991915291419 ) ) ;
#3800=CARTESIAN_POINT ( 'NONE',  ( -105.2107677708636544, -289.5361099034072936, -297.6573221304121262 ) ) ;
#3801=CARTESIAN_POINT ( 'NONE',  ( 24.65740365723694794, -286.4541666774916280, -224.8019473008992293 ) ) ;
#3803=CARTESIAN_POINT ( 'NONE',  ( 19.96044163558106277, -280.6031639379269791, -316.8880732669632607 ) ) ;
#3804=CARTESIAN_POINT ( 'NONE',  ( 33.00363917865989549, -289.1027651777063170, -246.6461708482359541 ) ) ;
#3805=CARTESIAN_POINT ( 'NONE',  ( -18.57760694158791992, -281.2860604328961927, -341.6784285630788531 ) ) ;
#3806=CARTESIAN_POINT ( 'NONE',  ( -104.9019450405615430, -280.2533242400683662, -241.4326409383732823 ) ) ;
#3807=CARTESIAN_POINT ( 'NONE',  ( 34.62945368840601645, -288.1547741847199404, -243.6595593979861292 ) ) ;
#3808=CARTESIAN_POINT ( 'NONE',  ( -92.76923378251689201, -278.3673619375146586, -317.9612960788221585 ) ) ;
#3809=CARTESIAN_POINT ( 'NONE',  ( -112.5322414616984901, -289.5320085612436856, -255.6507507476649721 ) ) ;
#3811=CARTESIAN_POINT ( 'NONE',  ( -113.4379889354556070, -285.2167501435198460, -281.3908560555238410 ) ) ;
#3812=CARTESIAN_POINT ( 'NONE',  ( -1.004161295595429104, -287.0137118053792733, -202.5443783457734810 ) ) ;
#3813=CARTESIAN_POINT ( 'NONE',  ( -33.49410224138745207, -283.1690883240081007, -343.2722227151212451 ) ) ;
#3815=CARTESIAN_POINT ( 'NONE',  ( -97.38415354343349861, -293.0393986255323284, -224.1317913308921845 ) ) ;
#3816=CARTESIAN_POINT ( 'NONE',  ( 26.09345564753667190, -291.6687573174892236, -227.4978217854600757 ) ) ;
#3817=CARTESIAN_POINT ( 'NONE',  ( -36.72207634974510881, -273.1188707359617638, -197.1159888817449257 ) ) ;
#3818=CARTESIAN_POINT ( 'NONE',  ( -111.4959257250324924, -295.6453885704456752, -290.7194974103967411 ) ) ;
#3819=CARTESIAN_POINT ( 'NONE',  ( -92.17623646728226561, -289.7302232938142197, -221.1093197897206721 ) ) ;
#3820=CARTESIAN_POINT ( 'NONE',  ( -8.861382141778378241, -292.9142792264262880, -338.6892246676347327 ) ) ;
#3821=CARTESIAN_POINT ( 'NONE',  ( -86.98672413512964852, -290.9665472029911939, -324.4902227632713334 ) ) ;
#3822=DIRECTION ( 'NONE',  ( 0.000000000000000000, 0.000000000000000000, 1.000000000000000000 ) ) ;
#3823=CARTESIAN_POINT ( 'NONE',  ( 35.67293339134257479, -291.7814474073047109, -288.2724381629643631 ) ) ;
#3824=CARTESIAN_POINT ( 'NONE',  ( 24.33859369159023345, -296.1311152283219030, -313.0511580319457039 ) ) ;
#3825=CARTESIAN_POINT ( 'NONE',  ( 12.32414570359500061, -289.2817760311842221, -324.2511521285316576 ) ) ;
#3826=CARTESIAN_POINT ( 'NONE',  ( 4.969041158637687694, -278.4632856510345391, -332.7166147122437678 ) ) ;
#3827=CARTESIAN_POINT ( 'NONE',  ( -72.67127316535380999, -276.3043180960522136, -338.3450783578011283 ) ) ;
#3828=CARTESIAN_POINT ( 'NONE',  ( -35.46651847218083731, -297.2722413285309813, -193.5228410401993244 ) ) ;
#3829=CARTESIAN_POINT ( 'NONE',  ( 17.26383780331741846, -274.4991361181947696, -320.3420922601056304 ) ) ;
#3830=CARTESIAN_POINT ( 'NONE',  ( -3.674848277866018087, -278.5797528103818195, -203.9552551387219239 ) ) ;
#3831=CARTESIAN_POINT ( 'NONE',  ( 21.79203441000850461, -276.1513377228506556, -226.8831701784761776 ) ) ;
#3832=CARTESIAN_POINT ( 'NONE',  ( -71.23353334215805432, -275.8919994566852552, -338.6090780963942848 ) ) ;
#3834=CARTESIAN_POINT ( 'NONE',  ( -102.1246206068893940, -273.6651385091302018, -236.3830957407453184 ) ) ;
#3836=CARTESIAN_POINT ( 'NONE',  ( -62.24440673204787089, -287.3944031294223009, -341.5377645544289180 ) ) ;
#3837=CARTESIAN_POINT ( 'NONE',  ( 33.83423658172637261, -275.1708802348304630, -254.0883783344873166 ) ) ;
#3838=CARTESIAN_POINT ( 'NONE',  ( -12.22372873399449311, -288.7343269669929100, -343.2049522237026622 ) ) ;
#3839=CARTESIAN_POINT ( 'NONE',  ( -30.69179918307676047, -300.1148906191218089, -195.0036787439324826 ) ) ;
#3840=CARTESIAN_POINT ( 'NONE',  ( -108.4408398538581366, -294.8561388163880110, -246.8530472998392327 ) ) ;
#3841=CARTESIAN_POINT ( 'NONE',  ( 31.88044968381650790, -280.3191656451151630, -236.8852224378985341 ) ) ;
#3843=CARTESIAN_POINT ( 'NONE',  ( -4.125849016030076477, -278.4899119336675426, -203.1034748114884678 ) ) ;
#3845=CARTESIAN_POINT ( 'NONE',  ( -108.4896135967199342, -289.5843662271626613, -252.2793800626216694 ) ) ;
#3848=CARTESIAN_POINT ( 'NONE',  ( -104.1806912062201889, -289.0031135144143377, -236.2234462952982312 ) ) ;
#3849=CARTESIAN_POINT ( 'NONE',  ( -54.39054924004955183, -275.3492675188937824, -198.6670143585344022 ) ) ;
#3850=CARTESIAN_POINT ( 'NONE',  ( 27.81215116149938282, -283.5041391352590381, -310.3811201814481819 ) ) ;
#3851=CARTESIAN_POINT ( 'NONE',  ( -111.6475788109127762, -270.8102793284238032, -256.3727456962960218 ) ) ;
#3852=CARTESIAN_POINT ( 'NONE',  ( -93.42207030925594324, -283.8890286302528239, -317.0943190321610814 ) ) ;
#3853=CARTESIAN_POINT ( 'NONE',  ( -46.26810626372915891, -275.3619658972887123, -197.3152817565799069 ) ) ;
#3854=CARTESIAN_POINT ( 'NONE',  ( 9.580829515692020237, -275.5195125063872297, -214.1621018541664228 ) ) ;
#3855=CARTESIAN_POINT ( 'NONE',  ( 22.67050588876224637, -284.1669401021530348, -315.3448459382437363 ) ) ;
#3856=CARTESIAN_POINT ( 'NONE',  ( -76.71872781989530665, -272.4316568420984481, -208.5252403431800019 ) ) ;
#3859=CARTESIAN_POINT ( 'NONE',  ( 19.52824766555975344, -294.0919391089947794, -322.3503284480491970 ) ) ;
#3860=CARTESIAN_POINT ( 'NONE',  ( -107.7161797551716518, -286.2063611641913212, -295.4002116545882473 ) ) ;
#3862=CARTESIAN_POINT ( 'NONE',  ( 15.93645355044460921, -281.4702648963637444, -320.5744003001203737 ) ) ;
#3863=CARTESIAN_POINT ( 'NONE',  ( -119.3990491898856732, -282.0523547857346784, -270.3284710469131937 ) ) ;
#3864=CARTESIAN_POINT ( 'NONE',  ( -106.2052141782906318, -277.3089545510403013, -304.5686183027536913 ) ) ;
#3865=CARTESIAN_POINT ( 'NONE',  ( -111.5336455799082813, -289.1716553820066338, -252.9830959788331199 ) ) ;
#3866=CARTESIAN_POINT ( 'NONE',  ( -2.080041497264457195, -284.0965032753784385, -335.0850740678901047 ) ) ;
#3868=CARTESIAN_POINT ( 'NONE',  ( -87.76980426881645769, -279.5286494010926504, -324.5365766746646727 ) ) ;
#3869=CARTESIAN_POINT ( 'NONE',  ( -29.54127319221524317, -287.5743836886140912, -194.3495423381301350 ) ) ;
#3870=CARTESIAN_POINT ( 'NONE',  ( -49.49028958735146944, -281.8974109375523085, -196.3515752167647577 ) ) ;
#3871=CARTESIAN_POINT ( 'NONE',  ( 1.193582804254908591, -274.7185470624626191, -203.6822600330811781 ) ) ;
#3872=CARTESIAN_POINT ( 'NONE',  ( -107.5769756848989545, -277.9809490391822351, -302.0504314144416185 ) ) ;
#3873=CARTESIAN_POINT ( 'NONE',  ( -101.3932908513521056, -297.9599835026583037, -308.3928622960517600 ) ) ;
#3877=CARTESIAN_POINT ( 'NONE',  ( -110.0607289645893587, -271.0744741343257829, -248.1379112651184755 ) ) ;
#3878=CARTESIAN_POINT ( 'NONE',  ( -96.93952468164245317, -277.4699290209426863, -312.6449797877878609 ) ) ;
#3879=CARTESIAN_POINT ( 'NONE',  ( -46.84701685229932622, -275.1390719887108958, -194.3502130286888701 ) ) ;
#3880=CARTESIAN_POINT ( 'NONE',  ( 7.523633233885763438, -288.4334962818484200, -211.4314836240222917 ) ) ;
#3881=CARTESIAN_POINT ( 'NONE',  ( -111.6263444986069828, -297.8513360954940481, -287.8674849973318146 ) ) ;
#3882=CARTESIAN_POINT ( 'NONE',  ( -97.08804772726796273, -297.1113003231642438, -318.3233230924677741 ) ) ;
#3884=CARTESIAN_POINT ( 'NONE',  ( -102.7379058268482623, -293.0387598460442860, -233.8765426218124617 ) ) ;
#3885=CARTESIAN_POINT ( 'NONE',  ( -80.08159532274385128, -277.4719795939890901, -208.9336828837877249 ) ) ;
#3886=CARTESIAN_POINT ( 'NONE',  ( -8.715753501634367240, -282.3498201072318921, -201.6452582478680711 ) ) ;
#3887=CARTESIAN_POINT ( 'NONE',  ( -111.8282507846819698, -270.6444425313729312, -264.7655964034407248 ) ) ;
#3888=CARTESIAN_POINT ( 'NONE',  ( -41.47762777424248526, -284.9639896214721944, -346.0644372150130152 ) ) ;
#3889=CARTESIAN_POINT ( 'NONE',  ( -11.90187720279179651, -285.3115920806744725, -201.6076345574216191 ) ) ;
#3890=CARTESIAN_POINT ( 'NONE',  ( 181.7315844963778204, 252.7314447161878661, -166.3319146787848410 ) ) ;
#3891=ORIENTED_EDGE ( 'NONE', *, *, #55197, .F. ) ;
#3892=CARTESIAN_POINT ( 'NONE',  ( 19.53433387065772564, -286.5713760049341090, -224.5460630323287887 ) ) ;
#3894=CARTESIAN_POINT ( 'NONE',  ( -78.98031843224808313, -284.6792455678940996, -334.7638972312655596 ) ) ;
#3895=CARTESIAN_POINT ( 'NONE',  ( -109.1512911691190055, -273.0636955951828213, -256.8440481922058893 ) ) ;
#3896=CARTESIAN_POINT ( 'NONE',  ( 38.16807301947188336, -286.1840028699430150, -257.3887898171809070 ) ) ;
#3897=CARTESIAN_POINT ( 'NONE',  ( 37.10013944839366928, -282.2581906540859791, -251.6199137984777678 ) ) ;
#3899=CARTESIAN_POINT ( 'NONE',  ( -86.37415712152908043, -280.9062222552844901, -211.8240706576670789 ) ) ;
#3900=CARTESIAN_POINT ( 'NONE',  ( 35.59041867844874929, -282.1976164632449127, -295.1570721854247950 ) ) ;
#3901=CARTESIAN_POINT ( 'NONE',  ( 27.36219212280433055, -284.6237833571632905, -239.2376011013261916 ) ) ;
#3902=CARTESIAN_POINT ( 'NONE',  ( 6.097804300016943735, -58.55705473465773281, -354.8591203811397463 ) ) ;
#3904=CARTESIAN_POINT ( 'NONE',  ( 37.43522874238411902, -277.6041177106234272, -274.3864749951786166 ) ) ;
#3905=CARTESIAN_POINT ( 'NONE',  ( 189.1269273087761746, 271.5004129489445859, -139.4852769914478756 ) ) ;
#3906=CARTESIAN_POINT ( 'NONE',  ( 23.46775487827690654, -278.9808892367470889, -227.0707381497046811 ) ) ;
#3907=CARTESIAN_POINT ( 'NONE',  ( 23.98321471386222470, -294.7086033295246352, -225.4920993278231549 ) ) ;
#3908=CARTESIAN_POINT ( 'NONE',  ( -70.98508551709741710, -294.8569315755531193, -335.2751632507477666 ) ) ;
#3909=CARTESIAN_POINT ( 'NONE',  ( -72.13882231151022495, -291.1120482898492696, -201.7266562873833777 ) ) ;
#3911=CARTESIAN_POINT ( 'NONE',  ( -104.0970417118808768, -294.6399437678667255, -307.6490353800345474 ) ) ;
#3912=CARTESIAN_POINT ( 'NONE',  ( 35.54615633446665157, -286.1040052329445871, -282.0087430885778303 ) ) ;
#3913=CARTESIAN_POINT ( 'NONE',  ( 28.57260044242703145, -294.9558767396604253, -236.2118799550954407 ) ) ;
#3914=CARTESIAN_POINT ( 'NONE',  ( -107.8327192305908824, -286.1426761573477506, -249.3936192887715606 ) ) ;
#3916=CARTESIAN_POINT ( 'NONE',  ( 36.85207186405477842, -294.2454271874594269, -250.6100683830450180 ) ) ;
#3917=CARTESIAN_POINT ( 'NONE',  ( -107.8188564907485443, -284.7896946007451788, -289.6686294985610175 ) ) ;
#3918=CARTESIAN_POINT ( 'NONE',  ( -112.7455393479568500, -295.5168014389322479, -256.8603865158926283 ) ) ;
#3919=CARTESIAN_POINT ( 'NONE',  ( -112.7684182332622100, -291.5395922517828353, -255.6307074632259173 ) ) ;
#3920=CARTESIAN_POINT ( 'NONE',  ( -84.23381177032861444, -291.9193052115301157, -209.2967807060013570 ) ) ;
#3921=CARTESIAN_POINT ( 'NONE',  ( -21.12727545794537320, -289.0049481451823112, -341.5376059339846506 ) ) ;
#3924=CARTESIAN_POINT ( 'NONE',  ( -99.74693943026251475, -298.9892499639144603, -227.3744683607866079 ) ) ;
#3925=CARTESIAN_POINT ( 'NONE',  ( -111.4302628277299334, -271.5943354071937392, -250.6930690799671879 ) ) ;
#3926=CARTESIAN_POINT ( 'NONE',  ( 0.5318640914145956744, -279.6287387840284282, -207.6206613115326434 ) ) ;
#3929=CARTESIAN_POINT ( 'NONE',  ( 38.67395804321970587, -275.2126909379657604, -282.5758344602695615 ) ) ;
#3930=CARTESIAN_POINT ( 'NONE',  ( -70.76486760227054162, -296.0829234350040906, -204.6690761318453724 ) ) ;
#3931=CARTESIAN_POINT ( 'NONE',  ( -3.279958271336609332, -278.4577381665240523, -336.3206754745209537 ) ) ;
#3932=CARTESIAN_POINT ( 'NONE',  ( 16.35638309704997084, -272.9640199228561528, -219.0286924979402556 ) ) ;
#3933=CARTESIAN_POINT ( 'NONE',  ( -93.05577821529237781, -298.4338955351863660, -222.5602783544774752 ) ) ;
#3934=CARTESIAN_POINT ( 'NONE',  ( -86.31696427394523141, -298.4327590036571678, -215.8116030930952718 ) ) ;
#3936=CARTESIAN_POINT ( 'NONE',  ( -113.5110041914985430, -298.1973691151788444, -266.7932724350081344 ) ) ;
#3937=CARTESIAN_POINT ( 'NONE',  ( -109.4555446166864954, -270.8547586346160756, -248.3197336285120116 ) ) ;
#3938=CARTESIAN_POINT ( 'NONE',  ( 3.880696444029271053, -295.1319988853880432, -330.7316959887211851 ) ) ;
#3939=CARTESIAN_POINT ( 'NONE',  ( -44.33830144156664943, -290.5367903350182814, -197.0540205050876637 ) ) ;
#3942=CARTESIAN_POINT ( 'NONE',  ( 38.86236064766877263, -275.9117602386304497, -259.7560237114771553 ) ) ;
#3943=CARTESIAN_POINT ( 'NONE',  ( -63.09089416710570930, -298.0407648374106202, -201.9770537296492705 ) ) ;
#3944=CARTESIAN_POINT ( 'NONE',  ( 32.78430889520149805, -283.1730981371846951, -242.6371301171608650 ) ) ;
#3946=CARTESIAN_POINT ( 'NONE',  ( -44.39056898841063514, -281.8242437299555831, -346.5955736806773189 ) ) ;
#3947=CARTESIAN_POINT ( 'NONE',  ( 0.9890151541174989624, -275.9035728178853333, -337.0853642246066784 ) ) ;
#3949=CARTESIAN_POINT ( 'NONE',  ( -103.6274440919934534, -284.1679605102631285, -239.2765322247979043 ) ) ;
#3950=CARTESIAN_POINT ( 'NONE',  ( -6.237961062326914607, -280.6442960687672326, -338.7905403553558585 ) ) ;
#3951=CARTESIAN_POINT ( 'NONE',  ( 36.28808916097170822, -274.1432537918842627, -271.6129572846691644 ) ) ;
#3952=CARTESIAN_POINT ( 'NONE',  ( -110.2397754343363090, -280.3252676258772453, -288.0462152943991896 ) ) ;
#3955=CARTESIAN_POINT ( 'NONE',  ( -57.88612961976851068, -272.1911191981950537, -196.9280281509629447 ) ) ;
#3956=CARTESIAN_POINT ( 'NONE',  ( -97.32466134903762622, -279.9340385015618153, -315.6820441345582822 ) ) ;
#3957=DIRECTION ( 'NONE',  ( 0.000000000000000000, 0.000000000000000000, 1.000000000000000000 ) ) ;
#3958=CARTESIAN_POINT ( 'NONE',  ( -105.3930203544997397, -286.9016394110923898, -237.5231519892752203 ) ) ;
#3960=CARTESIAN_POINT ( 'NONE',  ( -32.59055472263807474, -286.9922305065118167, -345.2609619176300271 ) ) ;
#3962=CARTESIAN_POINT ( 'NONE',  ( -107.2521678640016063, -295.0502972760867237, -292.8787700620900409 ) ) ;
#3963=CARTESIAN_POINT ( 'NONE',  ( -15.51064158014850491, -286.9063134480295503, -341.3674231275247166 ) ) ;
#3965=CARTESIAN_POINT ( 'NONE',  ( -109.5346917680343779, -294.2904637160274888, -290.6877657296118969 ) ) ;
#3966=CARTESIAN_POINT ( 'NONE',  ( -66.90243596928769421, -284.1515985747753348, -200.0129079831128536 ) ) ;
#3967=CARTESIAN_POINT ( 'NONE',  ( -2.792420425637325287, -282.1169338827938304, -205.1333854750963610 ) ) ;
#3968=CARTESIAN_POINT ( 'NONE',  ( -83.28854091667598425, -281.9113829519091041, -330.9488113130627198 ) ) ;
#3969=CARTESIAN_POINT ( 'NONE',  ( -74.71590172187745793, -289.5645964093313296, -333.0828143797020289 ) ) ;
#3970=CARTESIAN_POINT ( 'NONE',  ( -109.7148629322869766, -280.1517723286212345, -257.0381969833500193 ) ) ;
#3971=CARTESIAN_POINT ( 'NONE',  ( 20.63764013512398421, -281.7281467063703531, -225.7201619882444845 ) ) ;
#3972=CARTESIAN_POINT ( 'NONE',  ( 37.99509383334434887, -289.5107615713391738, -268.6955023555037201 ) ) ;
#3974=CARTESIAN_POINT ( 'NONE',  ( -78.84155419291386124, -273.5092632704380549, -205.5015611493715255 ) ) ;
#3975=CARTESIAN_POINT ( 'NONE',  ( -111.9490725445499493, -292.4849238040270052, -274.0140372659323020 ) ) ;
#3977=CARTESIAN_POINT ( 'NONE',  ( 40.65961533371913106, -296.2662352645559167, -288.1317622949166548 ) ) ;
#3979=CARTESIAN_POINT ( 'NONE',  ( 36.15822021795626284, -273.3495455904300115, -254.5588239821648529 ) ) ;
#3981=CARTESIAN_POINT ( 'NONE',  ( -99.36929568534276314, -294.3585989404804195, -314.7108157338814749 ) ) ;
#3982=CARTESIAN_POINT ( 'NONE',  ( -87.39706624112145050, -272.6804916913363854, -217.0156240571391777 ) ) ;
#3983=CARTESIAN_POINT ( 'NONE',  ( 8.425533636345621247, -289.9324263097764742, -328.1198235085651618 ) ) ;
#3984=CARTESIAN_POINT ( 'NONE',  ( -38.88402848578563464, -284.8318691571317345, -344.3710476100683309 ) ) ;
#3985=CARTESIAN_POINT ( 'NONE',  ( -71.92196545920795359, -293.0293575898770086, -202.2084493069208122 ) ) ;
#3986=CARTESIAN_POINT ( 'NONE',  ( -79.33780129512977908, -292.8135564267675477, -206.3475995486332693 ) ) ;
#3987=CARTESIAN_POINT ( 'NONE',  ( 21.80595542779304452, -292.7866763501625655, -227.5548767595264223 ) ) ;
#3988=CARTESIAN_POINT ( 'NONE',  ( -99.78598614260957333, -287.1135753174981460, -228.8194305723173443 ) ) ;
#3989=CARTESIAN_POINT ( 'NONE',  ( -75.00978690769282764, -279.7313267816818438, -203.2037264096550189 ) ) ;
#3990=CARTESIAN_POINT ( 'NONE',  ( -68.94827795070665388, -293.5443281292814959, -339.0071891260435564 ) ) ;
#3991=CARTESIAN_POINT ( 'NONE',  ( -93.43299178725850140, -283.6652946230617545, -323.1323868274789106 ) ) ;
#3992=CARTESIAN_POINT ( 'NONE',  ( 21.33061767708065304, -278.1688001777686168, -316.5271972907961526 ) ) ;
#3994=CARTESIAN_POINT ( 'NONE',  ( 30.91033621190086578, -296.2662352645559167, -285.9065529553535612 ) ) ;
#3995=CARTESIAN_POINT ( 'NONE',  ( -67.24328213961942424, -275.5796630498039690, -339.9757779007239265 ) ) ;
#3997=CARTESIAN_POINT ( 'NONE',  ( -1.227036590058407928, -282.0667193128870167, -333.8726879463029604 ) ) ;
#3998=CARTESIAN_POINT ( 'NONE',  ( -64.61537948573912615, -280.9090724401610828, -198.7219689535120040 ) ) ;
#3999=CARTESIAN_POINT ( 'NONE',  ( 32.64543012981248893, -287.0149876187390419, -301.8987432983395252 ) ) ;
#4000=CARTESIAN_POINT ( 'NONE',  ( -33.47764100108386032, -293.8615673356368347, -196.4360509522435336 ) ) ;
#4001=CARTESIAN_POINT ( 'NONE',  ( 32.29699949344013277, -277.5512180778191009, -301.2947878019139694 ) ) ;
#4002=CARTESIAN_POINT ( 'NONE',  ( 37.73158758126069756, -276.6817748453760260, -255.6200275691118975 ) ) ;
#4003=CARTESIAN_POINT ( 'NONE',  ( -35.11976253066777787, -276.8567960983031639, -343.3272950637256713 ) ) ;
#4004=CARTESIAN_POINT ( 'NONE',  ( -61.12203803105138888, -299.7430216211606648, -199.3519198207216334 ) ) ;
#4005=CARTESIAN_POINT ( 'NONE',  ( -112.1410887091962394, -282.5809905160034532, -268.1072565408044284 ) ) ;
#4006=CARTESIAN_POINT ( 'NONE',  ( 23.96096623889392774, -292.5980329817888901, -223.7805658431922495 ) ) ;
#4007=CARTESIAN_POINT ( 'NONE',  ( 21.79729763385790520, -289.8038797943099780, -318.4339171177215917 ) ) ;
#4008=CARTESIAN_POINT ( 'NONE',  ( 35.51251759422262921, -292.5854358490628329, -278.9603921538848113 ) ) ;
#4009=ORIENTED_EDGE ( 'NONE', *, *, #24867, .F. ) ;
#4010=CARTESIAN_POINT ( 'NONE',  ( -50.44731205546880659, -290.4626793910574065, -195.0826401322508161 ) ) ;
#4011=CARTESIAN_POINT ( 'NONE',  ( -32.15154794809505745, -291.7861051528240068, -197.5120346829365019 ) ) ;
#4013=CARTESIAN_POINT ( 'NONE',  ( -65.32138313132958274, -290.4889601323397414, -341.8219205522011634 ) ) ;
#4014=CARTESIAN_POINT ( 'NONE',  ( -109.2338518354734731, -279.3780383111872538, -257.1168289755672163 ) ) ;
#4016=CARTESIAN_POINT ( 'NONE',  ( -112.0080249597404531, -295.2519638753410618, -287.9231737092022172 ) ) ;
#4017=CARTESIAN_POINT ( 'NONE',  ( -29.48161483590419607, -286.8006493789483784, -193.8658119456694351 ) ) ;
#4018=CARTESIAN_POINT ( 'NONE',  ( -18.19139214208549049, -286.6255765077052047, -195.7472626910281690 ) ) ;
#4019=CARTESIAN_POINT ( 'NONE',  ( -100.4172623272052931, -284.3806398051031010, -307.1518904666638718 ) ) ;
#4020=CARTESIAN_POINT ( 'NONE',  ( -84.28609762920955006, -219.3914707876369050, -352.4634555978751678 ) ) ;
#4021=CARTESIAN_POINT ( 'NONE',  ( 159.5856148316313750, 220.3251242856082968, -204.2681947999263912 ) ) ;
#4022=CARTESIAN_POINT ( 'NONE',  ( 152.6535939263449109, 205.0357462877106798, -214.3309654381289420 ) ) ;
#4024=AXIS2_PLACEMENT_3D ( 'NONE', #80863, #24026, #15073 ) ;
#4025=CARTESIAN_POINT ( 'NONE',  ( 19.13000027186423324, -274.0915920411455318, -223.8471546873101090 ) ) ;
#4026=CARTESIAN_POINT ( 'NONE',  ( -13.69865890452786061, -275.6583918228139964, -339.8063541832243004 ) ) ;
#4027=CARTESIAN_POINT ( 'NONE',  ( -40.43150215130466307, -297.5220758740396718, -193.4326384129933842 ) ) ;
#4028=CARTESIAN_POINT ( 'NONE',  ( 161.8949478297373048, 217.5625359936354926, -202.7765268075980316 ) ) ;
#4029=CARTESIAN_POINT ( 'NONE',  ( 37.69540036843609698, -274.4248344230874181, -285.2853205819436084 ) ) ;
#4030=CARTESIAN_POINT ( 'NONE',  ( -90.94576330318855639, -275.0383167652792054, -219.3074990926179169 ) ) ;
#4032=CARTESIAN_POINT ( 'NONE',  ( -100.9598543248765878, -274.1993811033202064, -227.4387219108742784 ) ) ;
#4034=CARTESIAN_POINT ( 'NONE',  ( -63.83736815365980988, -289.8994016073442594, -338.5032898712450447 ) ) ;
#4035=CARTESIAN_POINT ( 'NONE',  ( -95.45266302553322646, -296.6744096911716042, -320.6331262177190524 ) ) ;
#4036=CARTESIAN_POINT ( 'NONE',  ( -114.2764895211900580, -297.0539072336697473, -269.6093972280968956 ) ) ;
#4037=CARTESIAN_POINT ( 'NONE',  ( -28.89387161511191238, -295.1088963941198813, -342.9216773273358285 ) ) ;
#4039=CARTESIAN_POINT ( 'NONE',  ( -92.27005585177633407, -279.7495852344541163, -322.3224873393675125 ) ) ;
#4041=CARTESIAN_POINT ( 'NONE',  ( 35.27169297381365709, -280.7369771262673908, -244.7692610333076857 ) ) ;
#4043=CARTESIAN_POINT ( 'NONE',  ( -11.15876004124781495, -277.6435906317606168, -338.7560161592641066 ) ) ;
#4044=CARTESIAN_POINT ( 'NONE',  ( 36.92019660882584731, -277.5170706682662285, -286.5199641268273467 ) ) ;
#4045=CARTESIAN_POINT ( 'NONE',  ( -112.4030575602510424, -276.6644657056460801, -263.1457901575126925 ) ) ;
#4046=CARTESIAN_POINT ( 'NONE',  ( -43.49355164788299533, -274.4648378832227422, -197.5082821846793024 ) ) ;
#4047=CARTESIAN_POINT ( 'NONE',  ( -98.40696098134409908, -271.6011207919544290, -229.0179435390359117 ) ) ;
#4049=CARTESIAN_POINT ( 'NONE',  ( -109.1324868316131642, -278.8933834816829744, -257.1292266207890975 ) ) ;
#4050=CARTESIAN_POINT ( 'NONE',  ( 21.10140636523384217, -286.9064663761558336, -319.7342035411035681 ) ) ;
#4051=CARTESIAN_POINT ( 'NONE',  ( 20.29705258445983773, -276.8896176567656653, -222.3738817825212948 ) ) ;
#4053=CARTESIAN_POINT ( 'NONE',  ( -50.79115954333742877, -288.4254054342342215, -342.3275407985929064 ) ) ;
#4054=CARTESIAN_POINT ( 'NONE',  ( -108.1365484681044649, -283.5165483416020038, -300.5207354781006757 ) ) ;
#4055=CARTESIAN_POINT ( 'NONE',  ( 35.56914304497294665, -279.6264126878859884, -257.6338652318328286 ) ) ;
#4056=CARTESIAN_POINT ( 'NONE',  ( 20.14761920898719083, -279.4830995175145745, -224.4225385385279026 ) ) ;
#4057=CARTESIAN_POINT ( 'NONE',  ( -100.8248340219891475, -283.1584755640865865, -231.3887262345100169 ) ) ;
#4058=CARTESIAN_POINT ( 'NONE',  ( 36.50029055872439443, -289.7245242943254198, -283.7734164794053981 ) ) ;
#4059=CARTESIAN_POINT ( 'NONE',  ( -109.1500874426143781, -279.5579548379943162, -285.5494693523274350 ) ) ;
#4061=CARTESIAN_POINT ( 'NONE',  ( -76.15658909139186505, -293.5340424949073395, -206.1264115607340273 ) ) ;
#4062=CARTESIAN_POINT ( 'NONE',  ( -66.94671055470398358, -277.9093002762613196, -200.3788532812752692 ) ) ;
#4063=CARTESIAN_POINT ( 'NONE',  ( -70.49162088761256939, -278.1527132285085600, -335.5145938848217497 ) ) ;
#4064=CARTESIAN_POINT ( 'NONE',  ( -75.79751954597993802, -285.5639878300248142, -335.0061147293567387 ) ) ;
#4066=CARTESIAN_POINT ( 'NONE',  ( -97.00718836604771411, -291.8413187080085436, -316.7221330200372904 ) ) ;
#4067=CARTESIAN_POINT ( 'NONE',  ( -111.8656736841943911, -294.6660120775948144, -261.4807654072386640 ) ) ;
#4068=CARTESIAN_POINT ( 'NONE',  ( 18.24177169860236347, -286.0216536380135608, -217.2312243296136955 ) ) ;
#4069=CARTESIAN_POINT ( 'NONE',  ( -101.8127393148392059, -289.4390505371529230, -234.3406728086626742 ) ) ;
#4071=CARTESIAN_POINT ( 'NONE',  ( -6.081977584088528843, -275.3173350994387079, -336.8886847156738895 ) ) ;
#4072=CARTESIAN_POINT ( 'NONE',  ( 11.07958883707165221, -292.5128886719675734, -326.6305079970456404 ) ) ;
#4074=CARTESIAN_POINT ( 'NONE',  ( -94.18180535206808202, -289.7289409008695316, -219.4503117475313729 ) ) ;
#4075=CARTESIAN_POINT ( 'NONE',  ( -49.57397602170458129, -287.4938622409321169, -197.5298536357526302 ) ) ;
#4076=CARTESIAN_POINT ( 'NONE',  ( -72.72219355050258116, -287.7539575484923944, -337.6229474402345545 ) ) ;
#4077=EDGE_CURVE ( 'NONE', #11917, #53167, #12642, .T. ) ;
#4078=CARTESIAN_POINT ( 'NONE',  ( -60.17857700567269319, -287.1755000690762927, -200.4050462610182706 ) ) ;
#4080=CARTESIAN_POINT ( 'NONE',  ( -68.85373024178605306, -286.4297520551655793, -204.3200775937451112 ) ) ;
#4081=CARTESIAN_POINT ( 'NONE',  ( 37.79901751891349448, -295.4594404071306144, -264.6796259179565141 ) ) ;
#4082=CARTESIAN_POINT ( 'NONE',  ( -70.95269423249102658, -275.5720255812921096, -338.0339727869271087 ) ) ;
#4083=CARTESIAN_POINT ( 'NONE',  ( -1.473817414965842953, -276.9230220807195337, -338.4730793496436263 ) ) ;
#4084=CARTESIAN_POINT ( 'NONE',  ( -39.15220980889361613, -290.1094812653827830, -194.8100163439370931 ) ) ;
#4085=CARTESIAN_POINT ( 'NONE',  ( -84.56693291321538197, -279.4222895713034518, -209.4760689945764227 ) ) ;
#4086=CARTESIAN_POINT ( 'NONE',  ( -93.40984197675048506, -297.8440626786731400, -319.6379916073888694 ) ) ;
#4089=CARTESIAN_POINT ( 'NONE',  ( -94.57320003151176024, -276.0324729095927410, -317.6612810275421452 ) ) ;
#4090=CARTESIAN_POINT ( 'NONE',  ( 22.99824609884386106, -278.9442864648622731, -225.8179755173599688 ) ) ;
#4092=CARTESIAN_POINT ( 'NONE',  ( -1.608873715906876889, -272.9969432454428784, -202.9380294246406038 ) ) ;
#4093=CARTESIAN_POINT ( 'NONE',  ( -99.30589279305291939, -297.5242994286335829, -310.3437424455297560 ) ) ;
#4094=CARTESIAN_POINT ( 'NONE',  ( -55.64179531581449112, -282.2027015615037158, -344.8366107637288565 ) ) ;
#4095=CARTESIAN_POINT ( 'NONE',  ( -63.17364631683722109, -298.6486375961428053, -201.7792268935036191 ) ) ;
#4096=CARTESIAN_POINT ( 'NONE',  ( -113.6304927380235199, -297.9482890320134629, -263.9286994929665298 ) ) ;
#4097=CARTESIAN_POINT ( 'NONE',  ( -68.28767609271420724, -273.3008831616714929, -204.2079119657149135 ) ) ;
#4098=CARTESIAN_POINT ( 'NONE',  ( 26.53834025783352146, -295.0238672201796817, -230.9644721543005517 ) ) ;
#4099=CARTESIAN_POINT ( 'NONE',  ( 24.14348973896150952, -288.3360602956159937, -316.7138032504097964 ) ) ;
#4100=CARTESIAN_POINT ( 'NONE',  ( 33.02806802026004362, -274.0553942585200389, -298.5809362263261164 ) ) ;
#4101=CARTESIAN_POINT ( 'NONE',  ( -26.14665468220148625, -288.7466964752044305, -346.5429462748469405 ) ) ;
#4103=CARTESIAN_POINT ( 'NONE',  ( 32.89903587378962868, -286.3369763580445237, -249.5889153477106106 ) ) ;
#4104=CARTESIAN_POINT ( 'NONE',  ( -111.1979718964696247, -288.7195278131462146, -257.3130617650502359 ) ) ;
#4106=CARTESIAN_POINT ( 'NONE',  ( -68.16629546550866792, -198.4621125041185792, -363.1570911012638021 ) ) ;
#4107=CARTESIAN_POINT ( 'NONE',  ( 27.08177225225482232, -287.5304661620513684, -304.9304168731330833 ) ) ;
#4109=CARTESIAN_POINT ( 'NONE',  ( -113.9180873375829890, -285.5697025661181101, -264.2788542957584355 ) ) ;
#4110=CARTESIAN_POINT ( 'NONE',  ( 36.48119578051298362, -292.3457168723773520, -249.2656232489793808 ) ) ;
#4111=CARTESIAN_POINT ( 'NONE',  ( 3.377078620101252149, -282.1894655818741171, -205.8905600691232678 ) ) ;
#4112=CARTESIAN_POINT ( 'NONE',  ( 36.12146946061618991, -282.5971331870076142, -248.9492403676707113 ) ) ;
#4113=CARTESIAN_POINT ( 'NONE',  ( -64.05734815539319982, -283.2439246382484725, -338.2969270598796356 ) ) ;
#4114=CARTESIAN_POINT ( 'NONE',  ( 33.15005505654980311, -277.8861981994871257, -296.1229791198512089 ) ) ;
#4115=CARTESIAN_POINT ( 'NONE',  ( -107.1663718575286310, -296.1367403650606320, -302.8190171424707273 ) ) ;
#4116=CARTESIAN_POINT ( 'NONE',  ( -3.895108466936783032, -275.8180782213758562, -204.9056516308431810 ) ) ;
#4117=CARTESIAN_POINT ( 'NONE',  ( -94.68762819549425558, -289.2355056356366845, -222.5573747271971285 ) ) ;
#4118=CARTESIAN_POINT ( 'NONE',  ( -37.13499189490923413, -296.9751344645247286, -197.0491815705110525 ) ) ;
#4121=CARTESIAN_POINT ( 'NONE',  ( -105.4205781120815146, -286.0749260667905105, -300.4705943560637706 ) ) ;
#4122=CARTESIAN_POINT ( 'NONE',  ( -37.67378505188158044, -296.1358488637872028, -347.0643144774864481 ) ) ;
#4123=CARTESIAN_POINT ( 'NONE',  ( -107.4873929206173671, -284.9311557883818864, -290.9842884770891942 ) ) ;
#4125=CARTESIAN_POINT ( 'NONE',  ( -35.72850811834609885, -276.0911642997310196, -347.1219561182802522 ) ) ;
#4126=CARTESIAN_POINT ( 'NONE',  ( -112.2199138107177276, -291.4228324734360172, -252.8520945127737320 ) ) ;
#4127=CARTESIAN_POINT ( 'NONE',  ( -110.6853137216536851, -282.4494680301459084, -289.4131381243500982 ) ) ;
#4128=CARTESIAN_POINT ( 'NONE',  ( -73.42755987748770963, -291.9201075764639768, -202.3494939518758713 ) ) ;
#4129=CARTESIAN_POINT ( 'NONE',  ( -31.86553411512128164, -289.3145719985016058, -343.2272700366625600 ) ) ;
#4132=CARTESIAN_POINT ( 'NONE',  ( 179.7466012574299725, 251.0770343007640690, -164.2655899362252683 ) ) ;
#4133=CARTESIAN_POINT ( 'NONE',  ( 8.805032570909716583, -283.9522771636744665, -331.1327134209747101 ) ) ;
#4134=CARTESIAN_POINT ( 'NONE',  ( 21.27581636871891391, -279.6952119285918457, -317.1477375740089997 ) ) ;
#4136=CARTESIAN_POINT ( 'NONE',  ( 33.03517741311532774, -280.2020894803011402, -249.8350082299948838 ) ) ;
#4137=CARTESIAN_POINT ( 'NONE',  ( -37.13128573027449164, -276.7162712372314672, -347.3527415445742577 ) ) ;
#4138=CARTESIAN_POINT ( 'NONE',  ( -108.9895957406937157, -280.8312899120113002, -248.7600188987238425 ) ) ;
#4139=CARTESIAN_POINT ( 'NONE',  ( 186.7585022445316838, 260.8546661130829989, -152.0293674503833472 ) ) ;
#4140=CARTESIAN_POINT ( 'NONE',  ( 3.522310748714557516, -279.1645524513189685, -205.7328376492112056 ) ) ;
#4141=CARTESIAN_POINT ( 'NONE',  ( -107.7330614769566210, -282.2472148643521450, -295.3527209834237510 ) ) ;
#4142=CARTESIAN_POINT ( 'NONE',  ( -106.9521679608413649, -274.8013060087374129, -240.3170026231693726 ) ) ;
#4143=CARTESIAN_POINT ( 'NONE',  ( -93.98628086929754488, -296.3916493914846910, -316.5259833511778993 ) ) ;
#4145=CARTESIAN_POINT ( 'NONE',  ( -2.188920048612625902, -291.2125573395861693, -205.8059427533700898 ) ) ;
#4146=CARTESIAN_POINT ( 'NONE',  ( -31.44978770529064604, -277.6311453919358314, -347.0856882651813180 ) ) ;
#4147=CARTESIAN_POINT ( 'NONE',  ( -2.913658196528595923, -274.5206400460447753, -205.9894632830011290 ) ) ;
#4148=CARTESIAN_POINT ( 'NONE',  ( 39.24651482946023862, -274.4111064346867010, -265.4732363449367654 ) ) ;
#4150=CARTESIAN_POINT ( 'NONE',  ( -37.62384662711495764, -272.0484977391615757, -195.3490580416540752 ) ) ;
#4154=CARTESIAN_POINT ( 'NONE',  ( 34.53647105710715692, -282.8219959130820484, -284.8380436314721464 ) ) ;
#4155=CARTESIAN_POINT ( 'NONE',  ( 37.15655596374822522, -283.5019555704919298, -285.3272081728183593 ) ) ;
#4156=CARTESIAN_POINT ( 'NONE',  ( -98.18731870919012295, -284.4624293883412633, -229.8431791444158137 ) ) ;
#4157=CARTESIAN_POINT ( 'NONE',  ( -24.20702140016851089, -275.2816531584898030, -343.0348947746628028 ) ) ;
#4158=CARTESIAN_POINT ( 'NONE',  ( -65.76711976480913791, -285.2883568993897256, -338.9523532805414447 ) ) ;
#4159=CARTESIAN_POINT ( 'NONE',  ( -107.7850624035687019, -276.7460210517311339, -292.1756294858532783 ) ) ;
#4160=CARTESIAN_POINT ( 'NONE',  ( -0.4023431909508938253, -275.6353175274970795, -207.0241959188328451 ) ) ;
#4162=CARTESIAN_POINT ( 'NONE',  ( -86.70881855613100697, -280.1890482956134178, -211.4101285665891794 ) ) ;
#4163=ORIENTED_EDGE ( 'NONE', *, *, #48459, .F. ) ;
#4165=CARTESIAN_POINT ( 'NONE',  ( -33.80900922685039234, -287.9565731022641444, -194.6787185946306238 ) ) ;
#4166=CARTESIAN_POINT ( 'NONE',  ( -15.55446817405715620, -293.9601632847988526, -340.2564994466360986 ) ) ;
#4167=CARTESIAN_POINT ( 'NONE',  ( -105.9094572422793590, -290.3508329957741694, -235.4331688118980708 ) ) ;
#4168=CARTESIAN_POINT ( 'NONE',  ( 28.57063116371966416, -285.3395244654289513, -236.5799861972809026 ) ) ;
#4169=CARTESIAN_POINT ( 'NONE',  ( -8.003490661816455187, -285.0189374764179888, -202.8730124851904293 ) ) ;
#4170=CARTESIAN_POINT ( 'NONE',  ( -110.1801013938541587, -288.6211012695011391, -283.4966163001510608 ) ) ;
#4171=CARTESIAN_POINT ( 'NONE',  ( -59.05101491641170242, -284.5443575837082903, -340.5275692681016722 ) ) ;
#4172=CARTESIAN_POINT ( 'NONE',  ( 36.52684549812997972, -273.3844072228177993, -257.3092040343902909 ) ) ;
#4173=CARTESIAN_POINT ( 'NONE',  ( -18.36138724680209933, -284.6924780804628767, -196.5082907733637398 ) ) ;
#4174=CARTESIAN_POINT ( 'NONE',  ( -92.21726406034277090, -299.2684638619484758, -219.1612401178895766 ) ) ;
#4175=CARTESIAN_POINT ( 'NONE',  ( 20.69137334903584957, -284.8945380587588261, -222.5888371770631124 ) ) ;
#4176=CARTESIAN_POINT ( 'NONE',  ( -38.36916137511170177, -280.9802185442484301, -197.1205897335820225 ) ) ;
#4177=CARTESIAN_POINT ( 'NONE',  ( -77.14350140077200990, -291.5840230152290360, -334.1858022588729114 ) ) ;
#4180=CARTESIAN_POINT ( 'NONE',  ( -32.08776164674274156, -296.9065414848801652, -345.7512453865664384 ) ) ;
#4181=CARTESIAN_POINT ( 'NONE',  ( -38.35599340309022409, -278.0392828225816402, -195.3552326248492079 ) ) ;
#4182=CARTESIAN_POINT ( 'NONE',  ( 11.02509503695413784, -291.8990194406365504, -210.5866092699514525 ) ) ;
#4183=CARTESIAN_POINT ( 'NONE',  ( -109.5577762349642796, -295.1512399430864093, -255.0925855094758390 ) ) ;
#4184=CARTESIAN_POINT ( 'NONE',  ( 35.62734420842953398, -280.3571962879857438, -279.5363100645913619 ) ) ;
#4185=CARTESIAN_POINT ( 'NONE',  ( -29.82052890166939818, -272.2279485180540064, -196.3020457450574270 ) ) ;
#4186=CARTESIAN_POINT ( 'NONE',  ( 10.62596837776658809, -295.6879674950345134, -326.0418709839166240 ) ) ;
#4187=CARTESIAN_POINT ( 'NONE',  ( -85.33152481854862970, -293.9090924074130839, -210.2361428286348826 ) ) ;
#4188=CARTESIAN_POINT ( 'NONE',  ( -99.34676823814790225, -295.6267883916999040, -225.8855147573280249 ) ) ;
#4189=CARTESIAN_POINT ( 'NONE',  ( 38.22099402024237236, -291.6842995323007131, -261.8618256588219424 ) ) ;
#4190=CARTESIAN_POINT ( 'NONE',  ( -9.521413983935405057, -293.8481037876265987, -202.1790362693750467 ) ) ;
#4192=CARTESIAN_POINT ( 'NONE',  ( -77.35199403553258435, -292.3030660243553029, -209.1093579413192458 ) ) ;
#4194=CARTESIAN_POINT ( 'NONE',  ( -34.56536661339670502, -281.0375271304656621, -345.6651602215052890 ) ) ;
#4195=CARTESIAN_POINT ( 'NONE',  ( -77.94974150490634202, -295.6143802988760285, -331.0850701778412599 ) ) ;
#4196=CARTESIAN_POINT ( 'NONE',  ( -65.25218816925747944, -283.4069928950823396, -342.1388546935320392 ) ) ;
#4197=CARTESIAN_POINT ( 'NONE',  ( -52.91748554546068561, -282.9131172425765612, -345.8021939631918258 ) ) ;
#4198=CARTESIAN_POINT ( 'NONE',  ( 2.260736105578529109, -286.5201396416985062, -333.8565939625161150 ) ) ;
#4200=CARTESIAN_POINT ( 'NONE',  ( 27.70377035048882419, -280.5592194406066255, -310.3585126206784253 ) ) ;
#4201=CARTESIAN_POINT ( 'NONE',  ( 38.36756507663325522, -286.6301174334181496, -282.9147199469671818 ) ) ;
#4203=CARTESIAN_POINT ( 'NONE',  ( 33.39002088987867012, -294.8745263657532973, -249.1266023085734957 ) ) ;
#4204=CARTESIAN_POINT ( 'NONE',  ( 16.55260188110149144, -277.7297356807420670, -324.6015270113794031 ) ) ;
#4205=CARTESIAN_POINT ( 'NONE',  ( -24.86860773075179054, -279.8823871677609532, -198.4131544760020063 ) ) ;
#4206=CARTESIAN_POINT ( 'NONE',  ( -39.21381946646181405, -292.1959778550440774, -193.3708447783596114 ) ) ;
#4207=CARTESIAN_POINT ( 'NONE',  ( -22.04190996844411998, -280.9374547131282611, -344.3559192611696744 ) ) ;
#4208=CARTESIAN_POINT ( 'NONE',  ( 30.80010111909687964, -292.9702563063384559, -297.3345522005225803 ) ) ;
#4209=CARTESIAN_POINT ( 'NONE',  ( -112.2382565473547658, -294.4900537429583096, -275.1846851534240272 ) ) ;
#4212=CARTESIAN_POINT ( 'NONE',  ( -31.60377231116232011, -294.4855549584206642, -343.2471480796669994 ) ) ;
#4214=CARTESIAN_POINT ( 'NONE',  ( -67.68488546085839630, -283.1237833571631768, -207.2794874003663779 ) ) ;
#4215=CARTESIAN_POINT ( 'NONE',  ( -20.56176820114410120, -297.3161699555620316, -193.5990152263022992 ) ) ;
#4216=CARTESIAN_POINT ( 'NONE',  ( 31.26368744270867239, -280.1115420893711416, -302.6343871963346714 ) ) ;
#4217=CARTESIAN_POINT ( 'NONE',  ( -52.09470046452793213, -287.1824143256771436, -195.2361257388816114 ) ) ;
#4218=CARTESIAN_POINT ( 'NONE',  ( -56.06763861630832935, -289.1333197238089951, -340.9710225178475298 ) ) ;
#4219=CARTESIAN_POINT ( 'NONE',  ( -94.98335340706431396, -279.4297103065441092, -316.2958365410439683 ) ) ;
#4220=CARTESIAN_POINT ( 'NONE',  ( -111.7408124191033210, -294.4863248658026009, -277.0218771891208007 ) ) ;
#4221=CARTESIAN_POINT ( 'NONE',  ( -93.52809752311577540, -298.9888713023584046, -222.1642072319880583 ) ) ;
#4222=CARTESIAN_POINT ( 'NONE',  ( -96.42170391911561467, -276.7397615785031348, -313.9331218638359928 ) ) ;
#4224=CARTESIAN_POINT ( 'NONE',  ( -54.58630197043935794, -297.5031075614586484, -195.3386680176760422 ) ) ;
#4225=CARTESIAN_POINT ( 'NONE',  ( -97.71240946786747372, -291.8749898890026202, -313.9121415457458397 ) ) ;
#4226=CARTESIAN_POINT ( 'NONE',  ( 36.68770856708837869, -295.3811537351722336, -288.4736578652758112 ) ) ;
#4228=CARTESIAN_POINT ( 'NONE',  ( -70.01055816976165147, -290.1456800510612197, -335.7710074219556304 ) ) ;
#4230=CARTESIAN_POINT ( 'NONE',  ( -106.4253858110398454, -297.6378463578126343, -236.5860212583945668 ) ) ;
#4231=CARTESIAN_POINT ( 'NONE',  ( -112.9536128793037335, -288.7528828597431243, -265.5502835054620618 ) ) ;
#4232=CARTESIAN_POINT ( 'NONE',  ( -101.5344022653336111, -297.4447039228560357, -227.8513359639053419 ) ) ;
#4234=CARTESIAN_POINT ( 'NONE',  ( -113.4195521062967060, -291.9895813127763518, -276.9135001440978385 ) ) ;
#4235=CARTESIAN_POINT ( 'NONE',  ( -2.602324593224680793, -291.1233781216987495, -342.4248175857292154 ) ) ;
#4236=CARTESIAN_POINT ( 'NONE',  ( -101.1864263408305931, -287.0781584895506739, -231.2254389232448943 ) ) ;
#4237=CARTESIAN_POINT ( 'NONE',  ( 24.58339754690349821, -272.9817730931796973, -228.3225214590135863 ) ) ;
#4238=CARTESIAN_POINT ( 'NONE',  ( -91.25609276290481375, -275.1983037933019318, -219.0145704904673778 ) ) ;
#4239=CARTESIAN_POINT ( 'NONE',  ( -100.0680832594036218, -288.0883092018522120, -310.4449683020284283 ) ) ;
#4240=CARTESIAN_POINT ( 'NONE',  ( -48.29167134814407802, -279.0503558092549952, -345.3834968706803465 ) ) ;
#4242=CARTESIAN_POINT ( 'NONE',  ( 19.67601529265115445, -280.9081409778063403, -224.7762506667461082 ) ) ;
#4243=CARTESIAN_POINT ( 'NONE',  ( 23.77230217607897700, -280.3443105839075429, -230.1578303610482408 ) ) ;
#4244=CARTESIAN_POINT ( 'NONE',  ( 37.88186786092692415, -276.8192925845438594, -285.2911993525877961 ) ) ;
#4245=CARTESIAN_POINT ( 'NONE',  ( 38.03210091993377517, -280.5198121281973158, -284.1013343015498549 ) ) ;
#4246=CARTESIAN_POINT ( 'NONE',  ( -49.04336257823442224, -154.3693876292917935, -362.0194686267980160 ) ) ;
#4247=CARTESIAN_POINT ( 'NONE',  ( 28.89897917431056129, -276.9998969056514966, -309.1553523223985280 ) ) ;
#4250=CARTESIAN_POINT ( 'NONE',  ( -95.51182510166704276, -274.7442099589068789, -220.9553241550526650 ) ) ;
#4251=CARTESIAN_POINT ( 'NONE',  ( 35.77081079830085031, -295.8376638359844719, -253.6410175316879361 ) ) ;
#4255=CARTESIAN_POINT ( 'NONE',  ( 19.74728301808315578, -287.9840996634037538, -224.3512985151637338 ) ) ;
#4256=CARTESIAN_POINT ( 'NONE',  ( 24.70455110511624142, -288.7237657098153818, -226.4725704908159685 ) ) ;
#4257=CARTESIAN_POINT ( 'NONE',  ( -58.72686164203720693, -288.6846035173604719, -340.3179858515813407 ) ) ;
#4258=CARTESIAN_POINT ( 'NONE',  ( -23.79057737923814742, -285.7283635367068086, -194.5712588073002109 ) ) ;
#4260=CARTESIAN_POINT ( 'NONE',  ( 23.22985545500804960, -280.5333187678874651, -312.5218469854566479 ) ) ;
#4261=CARTESIAN_POINT ( 'NONE',  ( 35.50071217969385629, -289.5990877771174041, -284.7394628909108860 ) ) ;
#4262=CARTESIAN_POINT ( 'NONE',  ( -76.51189502661767960, -282.0660008204415021, -332.8426557925588440 ) ) ;
#4263=CARTESIAN_POINT ( 'NONE',  ( -65.01724975514589744, -280.9980117507555519, -202.2780258716403523 ) ) ;
#4264=CARTESIAN_POINT ( 'NONE',  ( -43.20578305953556963, -277.6205470209709461, -343.1869442604946130 ) ) ;
#4265=CARTESIAN_POINT ( 'NONE',  ( -88.37348079797668277, -290.1504330764801693, -213.2317378068778453 ) ) ;
#4266=CARTESIAN_POINT ( 'NONE',  ( -114.1930572173051814, -285.3237382281208738, -272.8542162425276842 ) ) ;
#4267=CARTESIAN_POINT ( 'NONE',  ( -91.86380583107865050, -285.7917353686707429, -216.0760657778604639 ) ) ;
#4268=CARTESIAN_POINT ( 'NONE',  ( 15.82731910058799585, -282.4396211179411580, -320.4545988898785254 ) ) ;
#4270=CARTESIAN_POINT ( 'NONE',  ( 145.2857639756989272, -299.5541904835127980, -192.9639945212225882 ) ) ;
#4271=CARTESIAN_POINT ( 'NONE',  ( -107.2369079515141124, -292.7905245998764485, -241.1213265772720149 ) ) ;
#4272=CARTESIAN_POINT ( 'NONE',  ( -30.72313024643193913, -290.8188571003982474, -194.0886686684267772 ) ) ;
#4273=CARTESIAN_POINT ( 'NONE',  ( 35.87839481415820586, -274.5912753839438096, -268.8690911606510667 ) ) ;
#4274=CARTESIAN_POINT ( 'NONE',  ( -44.79401450493713810, -294.4925861155777511, -346.9505620046683703 ) ) ;
#4275=CARTESIAN_POINT ( 'NONE',  ( -104.1770757972027326, -289.4471480319974717, -239.3169509027828497 ) ) ;
#4276=CARTESIAN_POINT ( 'NONE',  ( -89.22800780922275976, -294.0339188043994341, -323.2137024254167841 ) ) ;
#4277=CARTESIAN_POINT ( 'NONE',  ( -100.6386522667229855, -291.2485799324754225, -307.6179672432508028 ) ) ;
#4279=CARTESIAN_POINT ( 'NONE',  ( -112.2524175955854844, -292.5053411541834976, -274.0196770573660388 ) ) ;
#4280=CARTESIAN_POINT ( 'NONE',  ( -5.360478627843927590, -290.4718106534627964, -202.3373728463376438 ) ) ;
#4281=CARTESIAN_POINT ( 'NONE',  ( 37.60692213002425177, -295.6027232527513320, -274.2868913662403543 ) ) ;
#4282=CARTESIAN_POINT ( 'NONE',  ( -37.29271205320124238, -286.9939975706553810, -197.1133604448681638 ) ) ;
#4283=CARTESIAN_POINT ( 'NONE',  ( -16.26216608198313907, -276.3030766908516398, -197.9601632865850718 ) ) ;
#4284=CARTESIAN_POINT ( 'NONE',  ( -12.01203535027179825, -275.5247400301428229, -342.7107126001876622 ) ) ;
#4285=CARTESIAN_POINT ( 'NONE',  ( -36.53244849369291813, -297.2592142849998709, -193.5227000370792609 ) ) ;
#4286=CARTESIAN_POINT ( 'NONE',  ( 20.80483173727489188, -274.4293722689355945, -316.1740407382618514 ) ) ;
#4287=CARTESIAN_POINT ( 'NONE',  ( -39.72327999011758237, -278.1018875852079191, -195.9464540011245788 ) ) ;
#4288=CARTESIAN_POINT ( 'NONE',  ( -54.31819140029412551, -275.0342719877373838, -198.9543308562912500 ) ) ;
#4289=CARTESIAN_POINT ( 'NONE',  ( -79.79754388434909629, -276.0152815932032127, -333.7013552730261381 ) ) ;
#4291=CARTESIAN_POINT ( 'NONE',  ( -107.2964998494803126, -273.4861947032821377, -248.9692968721127215 ) ) ;
#4293=CARTESIAN_POINT ( 'NONE',  ( 22.81363351863807054, -286.1898352083263148, -315.7455056044452704 ) ) ;
#4294=CARTESIAN_POINT ( 'NONE',  ( 0.6142787894519449177, -274.4069187278359436, -208.0045331745921544 ) ) ;
#4295=CARTESIAN_POINT ( 'NONE',  ( -6.919925778501975877, -288.6638310299311456, -341.1108912274279987 ) ) ;
#4296=CARTESIAN_POINT ( 'NONE',  ( -111.5227320609347288, -289.9611542323395383, -290.9261074780434910 ) ) ;
#4297=CARTESIAN_POINT ( 'NONE',  ( -4.335954344953206530, -300.4432659257108753, -194.9948368513721562 ) ) ;
#4298=CARTESIAN_POINT ( 'NONE',  ( 15.59562159072019583, -292.3014939920101938, -323.3269408233277318 ) ) ;
#4300=CARTESIAN_POINT ( 'NONE',  ( 27.72008475687179185, -280.2118207979277145, -229.3820127615050524 ) ) ;
#4301=ADVANCED_FACE ( 'NONE', ( #44761 ), #59459, .F. ) ;
#4303=CARTESIAN_POINT ( 'NONE',  ( -112.0563281125624258, -276.6431129019024979, -263.2641419807241050 ) ) ;
#4305=CARTESIAN_POINT ( 'NONE',  ( -92.72137645607988077, -288.6633476063824446, -318.6057721245113044 ) ) ;
#4308=CARTESIAN_POINT ( 'NONE',  ( -41.68383955003493924, -289.9974237814847697, -195.4357007680625316 ) ) ;
#4309=CARTESIAN_POINT ( 'NONE',  ( -32.66619857750620071, -275.6322390957025164, -196.8036057870655497 ) ) ;
#4310=CARTESIAN_POINT ( 'NONE',  ( -19.04178497067908182, -284.2464920273695839, -344.6027149983022468 ) ) ;
#4311=CARTESIAN_POINT ( 'NONE',  ( -15.38253172874556185, -296.3458519441296630, -195.0132753957137766 ) ) ;
#4312=CARTESIAN_POINT ( 'NONE',  ( -48.32868293023025785, -283.1958957875103238, -342.5295751429100619 ) ) ;
#4313=CARTESIAN_POINT ( 'NONE',  ( 22.75159493093351415, -276.3890078506522059, -227.8637798803263195 ) ) ;
#4314=CARTESIAN_POINT ( 'NONE',  ( 13.60178376479612794, -275.5911607936069458, -217.8505173805758091 ) ) ;
#4315=CARTESIAN_POINT ( 'NONE',  ( -11.37006930069944310, -284.7141020945844616, -340.7759129648206908 ) ) ;
#4317=CARTESIAN_POINT ( 'NONE',  ( -39.16220003467072530, -297.0875296385581805, -197.1360045099840477 ) ) ;
#4319=CARTESIAN_POINT ( 'NONE',  ( 204.4793297709846911, 295.2867319150298613, -54.00000000005014300 ) ) ;
#4320=CARTESIAN_POINT ( 'NONE',  ( 38.07015933274296771, -293.5800473194682354, -285.9191209774903655 ) ) ;
#4321=CARTESIAN_POINT ( 'NONE',  ( -84.71067997099605407, -287.3759808388974761, -212.6048904755965623 ) ) ;
#4323=CARTESIAN_POINT ( 'NONE',  ( -19.11405058567864046, -274.3380690714489560, -350.3683826091709648 ) ) ;
#4324=CARTESIAN_POINT ( 'NONE',  ( -113.1415552914096025, -277.5915202344523891, -282.9524156863793110 ) ) ;
#4325=CARTESIAN_POINT ( 'NONE',  ( -99.23253275600042400, -288.3564317357208324, -314.8353118505963835 ) ) ;
#4326=CARTESIAN_POINT ( 'NONE',  ( -87.38560458511349793, -285.2851078335249895, -324.5263425455733568 ) ) ;
#4327=CARTESIAN_POINT ( 'NONE',  ( -26.85610241278956067, -278.6771306295833597, -343.6279334750709040 ) ) ;
#4328=CARTESIAN_POINT ( 'NONE',  ( -110.3683287282665191, -286.2640424177569685, -247.6947197772464904 ) ) ;
#4329=CARTESIAN_POINT ( 'NONE',  ( -57.67936274330781998, -281.7897016535160901, -198.1712286255379638 ) ) ;
#4330=CARTESIAN_POINT ( 'NONE',  ( -24.16169608688228010, -274.3825450011969451, -194.4433407492400647 ) ) ;
#4331=CARTESIAN_POINT ( 'NONE',  ( -65.09705353670513261, -277.2381374406559189, -342.2410803135458082 ) ) ;
#4332=CARTESIAN_POINT ( 'NONE',  ( -38.33750351381376476, -296.9848841524737963, -344.7944611630506984 ) ) ;
#4333=CARTESIAN_POINT ( 'NONE',  ( 151.9709352735115147, -299.5541904835127980, -192.9639945212225882 ) ) ;
#4335=CARTESIAN_POINT ( 'NONE',  ( -29.20084367881113252, -296.2926237717836671, -194.5988578826594164 ) ) ;
#4336=CARTESIAN_POINT ( 'NONE',  ( -8.720343734134340608, -276.1749290462664135, -337.5967390545733906 ) ) ;
#4337=CARTESIAN_POINT ( 'NONE',  ( -40.44158779905904311, -299.0938404527728949, -193.6809872192189346 ) ) ;
#4338=CARTESIAN_POINT ( 'NONE',  ( 34.36481372306668902, -289.0730028061952339, -251.9756347728458366 ) ) ;
#4339=CARTESIAN_POINT ( 'NONE',  ( -113.6175786899859190, -298.1173755723638692, -266.7872336141744540 ) ) ;
#4340=CARTESIAN_POINT ( 'NONE',  ( -88.32963576417394336, -296.9525763058929897, -327.6007515792217646 ) ) ;
#4341=CARTESIAN_POINT ( 'NONE',  ( -108.6925730765285181, -292.2585448293478976, -293.0951522366988229 ) ) ;
#4342=CARTESIAN_POINT ( 'NONE',  ( -88.77258847826377064, -277.3284009994634971, -215.9306094870748041 ) ) ;
#4343=CARTESIAN_POINT ( 'NONE',  ( -111.3325675027123651, -280.3608082087097273, -278.9803645532674068 ) ) ;
#4344=CARTESIAN_POINT ( 'NONE',  ( -75.93673604751245421, -295.6126749478929128, -206.6481063102666553 ) ) ;
#4345=CARTESIAN_POINT ( 'NONE',  ( -35.89857773759159443, -284.8946778257179062, -346.1250828407030440 ) ) ;
#4346=CARTESIAN_POINT ( 'NONE',  ( 18.01861155572832018, -285.7902995542362987, -222.3042561985201644 ) ) ;
#4347=CARTESIAN_POINT ( 'NONE',  ( 104.7134020687092288, 115.3893350944124023, -282.6128408094983797 ) ) ;
#4349=CARTESIAN_POINT ( 'NONE',  ( 15.04762028614208980, -286.4836426377549401, -219.4941680710666958 ) ) ;
#4351=CARTESIAN_POINT ( 'NONE',  ( 30.44214174502560866, -282.1654325912812169, -234.3753410823629508 ) ) ;
#4352=CARTESIAN_POINT ( 'NONE',  ( -93.79743264964480431, -273.5414747823694483, -224.0291723794845495 ) ) ;
#4353=CARTESIAN_POINT ( 'NONE',  ( -37.96374475585426467, -284.8394515829972420, -193.7607147140849122 ) ) ;
#4354=CARTESIAN_POINT ( 'NONE',  ( -28.26475800910624159, -281.1057687455061682, -194.0814854761429160 ) ) ;
#4356=CARTESIAN_POINT ( 'NONE',  ( -38.18186819212120042, -281.5619175406736190, -194.0590742811003793 ) ) ;
#4357=CARTESIAN_POINT ( 'NONE',  ( 38.40552625923182717, -282.0579204756764966, -284.1493837232054034 ) ) ;
#4358=CARTESIAN_POINT ( 'NONE',  ( -105.5795714935544112, -282.2666405000203440, -254.7536222014695397 ) ) ;
#4359=CARTESIAN_POINT ( 'NONE',  ( 45.61465944062903333, 12.28553147226080355, -332.1500543120573639 ) ) ;
#4361=CARTESIAN_POINT ( 'NONE',  ( -75.22288142050554427, -275.5466224907591481, -205.7639240263404758 ) ) ;
#4362=CARTESIAN_POINT ( 'NONE',  ( 201.5581938671040518, 293.7308772661893386, -83.16477369446880630 ) ) ;
#4363=CARTESIAN_POINT ( 'NONE',  ( 29.61557273233616883, -280.0108887494052965, -303.4718305634746685 ) ) ;
#4364=CARTESIAN_POINT ( 'NONE',  ( 38.23175922701547336, -295.4187360515148839, -278.7602937214786607 ) ) ;
#4365=CARTESIAN_POINT ( 'NONE',  ( -10.46022511962803314, -294.0404835468467013, -338.3411074621490684 ) ) ;
#4366=CARTESIAN_POINT ( 'NONE',  ( -74.64356818023807705, -291.0770540033107636, -203.0699778292946860 ) ) ;
#4368=CARTESIAN_POINT ( 'NONE',  ( -110.6552176378702228, -294.8541593320919674, -291.9418012946524073 ) ) ;
#4369=CARTESIAN_POINT ( 'NONE',  ( 34.47493497500671111, -286.1737906604378736, -287.3555682555879685 ) ) ;
#4370=CARTESIAN_POINT ( 'NONE',  ( 24.35486496336018902, -294.8487427027795320, -229.0767464079922036 ) ) ;
#4371=CARTESIAN_POINT ( 'NONE',  ( -100.0387176662299851, -286.3932823897014259, -231.9192731867592840 ) ) ;
#4373=CARTESIAN_POINT ( 'NONE',  ( 31.96834765718888249, -294.0677181543535994, -237.2385729010899524 ) ) ;
#4374=CARTESIAN_POINT ( 'NONE',  ( 33.38466208303379545, -282.2867953956458109, -288.7349995409943517 ) ) ;
#4375=CARTESIAN_POINT ( 'NONE',  ( -109.4717886956513269, -295.6743550546011079, -244.5685019611752864 ) ) ;
#4376=CARTESIAN_POINT ( 'NONE',  ( -99.73316204540834917, -290.7590045266941274, -315.2330078204165034 ) ) ;
#4377=CARTESIAN_POINT ( 'NONE',  ( -68.30975204457119787, -292.1485224526916227, -199.9158975258618796 ) ) ;
#4378=CARTESIAN_POINT ( 'NONE',  ( -8.216541390353109264, -288.8266213144314634, -337.3533770767477336 ) ) ;
#4381=CARTESIAN_POINT ( 'NONE',  ( -85.59020269727244568, -297.5719576801733979, -328.7767620998354801 ) ) ;
#4382=CARTESIAN_POINT ( 'NONE',  ( 30.26323651991097208, -297.5666936174177977, -193.8689913825462554 ) ) ;
#4383=CARTESIAN_POINT ( 'NONE',  ( -16.84441383036666195, -279.3822257687527895, -200.0527279998552501 ) ) ;
#4385=CARTESIAN_POINT ( 'NONE',  ( 37.53052916771648029, -275.2821372374443172, -288.1287512367670729 ) ) ;
#4387=CARTESIAN_POINT ( 'NONE',  ( -52.76144917968251491, -296.3309848438457834, -198.2466920969861235 ) ) ;
#4388=CARTESIAN_POINT ( 'NONE',  ( -18.68400137620172430, -278.6697342516281992, -342.2134370463454047 ) ) ;
#4389=CARTESIAN_POINT ( 'NONE',  ( 34.71373914236907865, -273.4600155537742694, -252.5039302194523998 ) ) ;
#4390=CARTESIAN_POINT ( 'NONE',  ( -71.09984203453312546, -296.7131203023845956, -335.5481651650862887 ) ) ;
#4391=CARTESIAN_POINT ( 'NONE',  ( -97.14282222425553925, -298.2214131598252038, -227.9576762577838451 ) ) ;
#4393=CARTESIAN_POINT ( 'NONE',  ( -106.4323516233798017, -297.7366112216848251, -302.5002263921336976 ) ) ;
#4394=CARTESIAN_POINT ( 'NONE',  ( -93.83628602626684767, -271.2622846344066829, -220.4936078306820946 ) ) ;
#4395=CARTESIAN_POINT ( 'NONE',  ( 6.731104131827689407, -293.3213210597814964, -212.0389044399694569 ) ) ;
#4396=CARTESIAN_POINT ( 'NONE',  ( -107.9556217973475611, -289.3992553413693258, -249.6029152947801322 ) ) ;
#4398=CARTESIAN_POINT ( 'NONE',  ( -18.57106110723369596, -274.7798704578709135, -195.6925283120649510 ) ) ;
#4399=CARTESIAN_POINT ( 'NONE',  ( -92.01956818916413283, -273.4098560835121248, -221.9944895202328041 ) ) ;
#4400=CARTESIAN_POINT ( 'NONE',  ( 17.93608662617683791, -282.8191428185303380, -219.1481011331267439 ) ) ;
#4401=CARTESIAN_POINT ( 'NONE',  ( 17.46125741984589652, -280.9743632908815698, -323.8215731871285357 ) ) ;
#4402=CARTESIAN_POINT ( 'NONE',  ( -106.2577176533503405, -277.4603495535039883, -304.5968569752323560 ) ) ;
#4403=CARTESIAN_POINT ( 'NONE',  ( -108.8801102275217971, -283.5468169684576196, -285.7457221856930119 ) ) ;
#4404=CARTESIAN_POINT ( 'NONE',  ( -0.06353451936536706757, -280.5572363385340395, -335.6474702640018108 ) ) ;
#4405=CARTESIAN_POINT ( 'NONE',  ( -2.619734573024061319, -273.0955980956678104, -205.4784544565968929 ) ) ;
#4406=CARTESIAN_POINT ( 'NONE',  ( -112.3822258285517961, -280.5359418150429178, -271.6364700943818775 ) ) ;
#4409=CARTESIAN_POINT ( 'NONE',  ( -36.18080114837113115, -296.3063621436284052, -194.3747869642731985 ) ) ;
#4410=CARTESIAN_POINT ( 'NONE',  ( -69.49315066435812582, -279.4743752187947621, -338.3186618418029639 ) ) ;
#4413=CARTESIAN_POINT ( 'NONE',  ( -104.4929723554661507, -286.0159826572646011, -305.1165235463112708 ) ) ;
#4415=CARTESIAN_POINT ( 'NONE',  ( 17.04995857286303362, -284.8273217527765269, -218.7039645495036098 ) ) ;
#4417=CARTESIAN_POINT ( 'NONE',  ( -106.3658192058961873, -295.0146595374200160, -295.4666403463573943 ) ) ;
#4418=CARTESIAN_POINT ( 'NONE',  ( -7.747493166749691795, -286.7998529430500412, -338.4972519408854055 ) ) ;
#4419=CARTESIAN_POINT ( 'NONE',  ( -115.8664652629750549, -267.0802710791712116, -295.7299871733738996 ) ) ;
#4420=CARTESIAN_POINT ( 'NONE',  ( -96.00004155097701641, -295.1944313328239105, -223.6256963487992380 ) ) ;
#4421=CARTESIAN_POINT ( 'NONE',  ( -87.28143286770665554, -283.8509541772170337, -212.5960267653878475 ) ) ;
#4422=CARTESIAN_POINT ( 'NONE',  ( 34.72599896870750058, -283.3597053636372038, -286.2572547625211996 ) ) ;
#4423=CARTESIAN_POINT ( 'NONE',  ( 37.79620794229941083, -279.6441498786120405, -258.6936146589770260 ) ) ;
#4424=CARTESIAN_POINT ( 'NONE',  ( -101.6431463815702898, -290.0796025691736304, -305.0272853527728216 ) ) ;
#4425=CARTESIAN_POINT ( 'NONE',  ( -104.9908093272758833, -280.3634047989733062, -241.3960883750020798 ) ) ;
#4426=CARTESIAN_POINT ( 'NONE',  ( 18.95381865755613404, -281.6935403467549577, -223.6146377524373747 ) ) ;
#4427=CARTESIAN_POINT ( 'NONE',  ( 25.74663376963620820, -288.9787978701504585, -229.1510594006102508 ) ) ;
#4429=CARTESIAN_POINT ( 'NONE',  ( -88.03637051047577700, -273.3660892892744982, -212.3329135229915039 ) ) ;
#4430=CARTESIAN_POINT ( 'NONE',  ( -91.77531105708733605, -291.8124940825813383, -321.5132671151195609 ) ) ;
#4432=CARTESIAN_POINT ( 'NONE',  ( 44.71564893372296723, -290.0519495502701943, -270.3284710469131937 ) ) ;
#4434=CARTESIAN_POINT ( 'NONE',  ( 37.78970020583974332, -273.5983726905885192, -273.9816781106921439 ) ) ;
#4436=CARTESIAN_POINT ( 'NONE',  ( -1.104756786260240764, -292.9794252604567077, -337.4081104003678888 ) ) ;
#4437=CARTESIAN_POINT ( 'NONE',  ( -96.14612360009986958, -296.6672362159974341, -226.9807065598966460 ) ) ;
#4438=CARTESIAN_POINT ( 'NONE',  ( 12.64013289151602493, -289.8605528047412463, -324.5832618425941973 ) ) ;
#4439=CARTESIAN_POINT ( 'NONE',  ( -69.42847045845644516, -285.2404528966351336, -337.0715356234218234 ) ) ;
#4440=CARTESIAN_POINT ( 'NONE',  ( -66.80513984946860262, -293.0988363928310605, -199.8592597562300170 ) ) ;
#4441=CARTESIAN_POINT ( 'NONE',  ( -105.5719445902916931, -292.3171037527162639, -235.6331031278305375 ) ) ;
#4442=CARTESIAN_POINT ( 'NONE',  ( -6.208915370107641607, -288.4613230956734924, -202.1139585754389714 ) ) ;
#4443=CARTESIAN_POINT ( 'NONE',  ( -3.659525067055291903, -280.6510602797544038, -201.1041918721884372 ) ) ;
#4444=CARTESIAN_POINT ( 'NONE',  ( -112.7974062411733343, -294.5700472872175055, -275.2219055470237663 ) ) ;
#4445=CARTESIAN_POINT ( 'NONE',  ( -65.25416720483168831, -283.2403397505250950, -342.1380851777612975 ) ) ;
#4446=CARTESIAN_POINT ( 'NONE',  ( 26.32316238324563074, -276.8949517552385942, -232.0824090322860798 ) ) ;
#4447=CARTESIAN_POINT ( 'NONE',  ( 30.91033621190086578, -284.2662352645559167, -285.9065529553535612 ) ) ;
#4449=CARTESIAN_POINT ( 'NONE',  ( -79.55791378705039563, -275.7550359584861894, -333.3376935469220257 ) ) ;
#4451=CARTESIAN_POINT ( 'NONE',  ( -67.81574721948939555, -282.9709276078943958, -336.7638355152207623 ) ) ;
#4452=CARTESIAN_POINT ( 'NONE',  ( -113.6820063142510548, -279.6698648228827437, -277.3104055157913876 ) ) ;
#4454=CARTESIAN_POINT ( 'NONE',  ( -40.79385542200716941, -285.0686119178861304, -193.6220391609869012 ) ) ;
#4455=CARTESIAN_POINT ( 'NONE',  ( -70.69719085749100884, -293.3661162045929132, -204.2900558275705691 ) ) ;
#4456=CARTESIAN_POINT ( 'NONE',  ( 37.93409632436373613, -277.0016873660071610, -258.4452096673913388 ) ) ;
#4457=ADVANCED_FACE ( 'NONE', ( #73661 ), #33869, .F. ) ;
#4458=CARTESIAN_POINT ( 'NONE',  ( 13.62340598719713824, -276.0633693407946794, -213.2302261979895661 ) ) ;
#4460=CARTESIAN_POINT ( 'NONE',  ( 31.26103323153933644, -275.7197067577321832, -295.4612537763394471 ) ) ;
#4461=CARTESIAN_POINT ( 'NONE',  ( -61.58357070194952598, -297.3678486710958850, -341.2140544523533663 ) ) ;
#4462=CARTESIAN_POINT ( 'NONE',  ( -111.9250100420552769, -282.4733336955501954, -276.4732621857104391 ) ) ;
#4463=CARTESIAN_POINT ( 'NONE',  ( -58.92868767960735710, -291.4469950619443352, -196.4710221652081259 ) ) ;
#4464=CARTESIAN_POINT ( 'NONE',  ( 38.77727348086906289, -289.0952099648609419, -265.8452818068897159 ) ) ;
#4465=CARTESIAN_POINT ( 'NONE',  ( 34.78978374617169322, -292.2996452670188887, -257.2040322935956169 ) ) ;
#4467=CARTESIAN_POINT ( 'NONE',  ( 19.94902896013509164, -291.4367960760712322, -219.7807011821576850 ) ) ;
#4468=CARTESIAN_POINT ( 'NONE',  ( 10.94796830920859598, -292.4086912619670215, -215.5196029281491406 ) ) ;
#4470=CARTESIAN_POINT ( 'NONE',  ( -67.91795386975798010, -290.5239002095117939, -340.6930823913618838 ) ) ;
#4471=CARTESIAN_POINT ( 'NONE',  ( -66.08193070137932068, -279.9986603228350077, -203.2200835328744404 ) ) ;
#4472=CARTESIAN_POINT ( 'NONE',  ( -113.9260196751459944, -295.4103946427232472, -275.3056861123669705 ) ) ;
#4473=CARTESIAN_POINT ( 'NONE',  ( -102.4366065921983733, -285.7403426842598151, -229.4225550025113023 ) ) ;
#4474=CARTESIAN_POINT ( 'NONE',  ( 9.794459312831646614, -287.0146167073599486, -209.5012234328941361 ) ) ;
#4475=CARTESIAN_POINT ( 'NONE',  ( -109.8932482333227370, -284.7706486160037116, -279.0650878718708441 ) ) ;
#4476=CARTESIAN_POINT ( 'NONE',  ( 121.4031722996727325, 149.7340073792644830, -263.5263209816934022 ) ) ;
#4477=CARTESIAN_POINT ( 'NONE',  ( -64.80429634339824929, -181.9903270017377963, -361.1305515816413845 ) ) ;
#4478=CARTESIAN_POINT ( 'NONE',  ( 199.9948420232396131, 290.8510889670257598, -82.40867480343716522 ) ) ;
#4479=CARTESIAN_POINT ( 'NONE',  ( 28.01010196456579138, -274.3039257947781380, -237.4712458382358022 ) ) ;
#4480=CARTESIAN_POINT ( 'NONE',  ( -37.82554206253664120, -275.9786430995062574, -343.6811398426501682 ) ) ;
#4481=CARTESIAN_POINT ( 'NONE',  ( -95.52044571051723665, -296.7411457569862137, -219.9352081809657591 ) ) ;
#4482=CARTESIAN_POINT ( 'NONE',  ( -75.69614664873641630, -208.8793829413635308, -354.1463231226688890 ) ) ;
#4483=CARTESIAN_POINT ( 'NONE',  ( 25.65125340681422372, -274.8149596424457286, -313.8715148012267946 ) ) ;
#4484=CARTESIAN_POINT ( 'NONE',  ( -33.76073202455672373, -299.9578568962608642, -196.1247607683412468 ) ) ;
#4485=CARTESIAN_POINT ( 'NONE',  ( -35.84592400321518113, -299.0116964481301238, -193.5961778596468719 ) ) ;
#4486=CARTESIAN_POINT ( 'NONE',  ( 35.05624986874159532, -287.9101389311853723, -260.1670901906311997 ) ) ;
#4487=CARTESIAN_POINT ( 'NONE',  ( -76.99012796964659344, -296.3715381577441121, -336.2421676807063022 ) ) ;
#4488=CARTESIAN_POINT ( 'NONE',  ( -91.59657762063839925, -297.7964346795590700, -215.8089853806745566 ) ) ;
#4489=CARTESIAN_POINT ( 'NONE',  ( 6.064644046955196544, -294.6115597621364373, -329.1172945606851954 ) ) ;
#4492=CARTESIAN_POINT ( 'NONE',  ( 37.31688773893979061, -277.6248027674322429, -282.3267299317424772 ) ) ;
#4494=CARTESIAN_POINT ( 'NONE',  ( -64.71456643181417689, -279.2119233047650937, -198.4004635590715679 ) ) ;
#4495=CARTESIAN_POINT ( 'NONE',  ( -35.09845810005103317, -277.9645489644905751, -343.5620490826685227 ) ) ;
#4496=CARTESIAN_POINT ( 'NONE',  ( 30.95448136916065707, -277.7470418235819807, -303.7917817540888450 ) ) ;
#4497=CARTESIAN_POINT ( 'NONE',  ( -107.1425661717945985, -276.2037867860376537, -298.7555875120523865 ) ) ;
#4498=CARTESIAN_POINT ( 'NONE',  ( -76.60257407051686585, -274.0034220950490180, -208.7447872019239412 ) ) ;
#4499=CARTESIAN_POINT ( 'NONE',  ( -84.87240992961781672, -294.2970994256663744, -326.6081637078360700 ) ) ;
#4501=CARTESIAN_POINT ( 'NONE',  ( -76.35402572753500294, -277.7560769139649892, -332.1217705409205223 ) ) ;
#4502=CARTESIAN_POINT ( 'NONE',  ( 22.01188697103727421, -286.8890492353381205, -318.6564642408707755 ) ) ;
#4503=CARTESIAN_POINT ( 'NONE',  ( -1.036491026389169123, -276.5341259920437551, -204.7192931778294565 ) ) ;
#4505=CARTESIAN_POINT ( 'NONE',  ( -53.45401580810245434, -288.4613374929169254, -341.7263406743113023 ) ) ;
#4506=CARTESIAN_POINT ( 'NONE',  ( -92.36659915629896034, -283.1629151545395757, -324.0786502548191379 ) ) ;
#4508=CARTESIAN_POINT ( 'NONE',  ( 34.75247382928597517, -279.5741336227684997, -253.6158470662637114 ) ) ;
#4509=CARTESIAN_POINT ( 'NONE',  ( 20.99406027203965053, -279.5004030761576814, -225.4818076967800096 ) ) ;
#4510=CARTESIAN_POINT ( 'NONE',  ( -111.8315654330356779, -282.6250756368986004, -270.8957085002210192 ) ) ;
#4512=CARTESIAN_POINT ( 'NONE',  ( -102.4856526618863768, -287.0491087079658428, -233.0922363453260573 ) ) ;
#4513=CARTESIAN_POINT ( 'NONE',  ( -102.5154956978138756, -280.2151364249276071, -236.4938788253674886 ) ) ;
#4515=CARTESIAN_POINT ( 'NONE',  ( 24.82058582463015028, -294.9835569248187994, -228.3073100600224166 ) ) ;
#4516=CARTESIAN_POINT ( 'NONE',  ( -111.8051715203650360, -276.5993514929936055, -285.5637239842043869 ) ) ;
#4518=CARTESIAN_POINT ( 'NONE',  ( 26.86024205217384164, -276.6813364551920245, -305.4241236169632998 ) ) ;
#4519=CARTESIAN_POINT ( 'NONE',  ( -106.5294224214257497, -286.1676952650918793, -299.8725170507947837 ) ) ;
#4521=CARTESIAN_POINT ( 'NONE',  ( -79.71251375888961377, -291.5397226768191672, -332.9865081745542170 ) ) ;
#4522=CARTESIAN_POINT ( 'NONE',  ( -56.01809048318838080, -293.2923762727940584, -343.0515620962855792 ) ) ;
#4523=CARTESIAN_POINT ( 'NONE',  ( -21.00830358765497508, -285.4537868550945632, -195.2786368205123040 ) ) ;
#4524=CARTESIAN_POINT ( 'NONE',  ( -100.3845383080752782, -289.4747267172832608, -231.9939318939462396 ) ) ;
#4526=CARTESIAN_POINT ( 'NONE',  ( -11.09345012332124192, -275.3875286777388851, -339.0071145870588225 ) ) ;
#4527=CARTESIAN_POINT ( 'NONE',  ( -0.1594568512881724687, -292.6919181326035755, -334.6719867168451970 ) ) ;
#4529=CARTESIAN_POINT ( 'NONE',  ( -103.9948696362666425, -289.5180309084092301, -233.2119222219740777 ) ) ;
#4530=CARTESIAN_POINT ( 'NONE',  ( -109.1485954315176343, -286.3752296681469147, -253.2710706312244611 ) ) ;
#4531=CARTESIAN_POINT ( 'NONE',  ( -29.10953442217389764, -287.1891884170248090, -345.9533682510087829 ) ) ;
#4533=CARTESIAN_POINT ( 'NONE',  ( -108.9430120123302004, -286.2004018803217491, -253.3177627417776421 ) ) ;
#4535=CARTESIAN_POINT ( 'NONE',  ( -37.29100371760605270, -286.8556005776840721, -197.1871922649171722 ) ) ;
#4536=CARTESIAN_POINT ( 'NONE',  ( 16.30063956946690240, -294.7885894542404799, -217.3640803795730960 ) ) ;
#4537=CARTESIAN_POINT ( 'NONE',  ( -79.44448346107091652, -275.6953074511906721, -333.1670029207481321 ) ) ;
#4538=CARTESIAN_POINT ( 'NONE',  ( 10.51623328085961440, -276.7453061544791240, -330.7231549890655629 ) ) ;
#4539=CARTESIAN_POINT ( 'NONE',  ( -19.69882036959028326, -290.3569827999576773, -196.8359410986647049 ) ) ;
#4540=CARTESIAN_POINT ( 'NONE',  ( -113.2991671191070822, -278.3942231741314117, -282.9889922418026345 ) ) ;
#4541=CARTESIAN_POINT ( 'NONE',  ( -78.84376550447035470, -297.5939536340089262, -332.4672736319399178 ) ) ;
#4544=CARTESIAN_POINT ( 'NONE',  ( 2.729830342520385589, -285.2870244002904201, -208.7533593551256388 ) ) ;
#4545=CARTESIAN_POINT ( 'NONE',  ( -105.4133529992866158, -276.2986472282068462, -300.1061580810805367 ) ) ;
#4546=CARTESIAN_POINT ( 'NONE',  ( 5.754406211532351101, -280.4684074942066445, -331.8064174026715136 ) ) ;
#4547=DIRECTION ( 'NONE',  ( 1.000000000000000000, 0.000000000000000000, 0.000000000000000000 ) ) ;
#4548=CARTESIAN_POINT ( 'NONE',  ( 37.27156885159967459, -273.8295064046976108, -254.3127855910245501 ) ) ;
#4549=CARTESIAN_POINT ( 'NONE',  ( -48.63175651213587258, -276.5481531940310447, -342.6374180482945349 ) ) ;
#4550=CARTESIAN_POINT ( 'NONE',  ( 36.22549824357571424, -295.0054804273252103, -265.2491425634210032 ) ) ;
#4551=CARTESIAN_POINT ( 'NONE',  ( -11.60010616948785156, -279.2998869186145043, -198.0636588701368623 ) ) ;
#4552=CARTESIAN_POINT ( 'NONE',  ( -39.68459460023145624, -296.0235152069855644, -343.5713980076945404 ) ) ;
#4553=CARTESIAN_POINT ( 'NONE',  ( -36.21040288203779056, -299.3812042098762731, -193.8540181952150192 ) ) ;
#4554=CARTESIAN_POINT ( 'NONE',  ( -79.72632205034507535, -297.2943201316504087, -210.9259110005620812 ) ) ;
#4555=CARTESIAN_POINT ( 'NONE',  ( -58.23589824656193059, -293.7824356898728979, -198.2760078724264474 ) ) ;
#4556=CARTESIAN_POINT ( 'NONE',  ( -30.88596906252780983, -286.2982626311953709, -193.6189267934908003 ) ) ;
#4557=CARTESIAN_POINT ( 'NONE',  ( 28.01822719600309242, -274.1986802453183714, -308.6806349260861566 ) ) ;
#4558=CARTESIAN_POINT ( 'NONE',  ( -69.35924035416215361, -289.2952204175426232, -340.4032300449738386 ) ) ;
#4559=CARTESIAN_POINT ( 'NONE',  ( -110.2179709872880267, -280.7411115577180567, -254.1502397022773607 ) ) ;
#4560=CARTESIAN_POINT ( 'NONE',  ( 8.116651766637280829, -287.4714484460505446, -327.7801626488054580 ) ) ;
#4561=CARTESIAN_POINT ( 'NONE',  ( -112.0129842500113142, -288.6489151959764285, -262.8122605209726430 ) ) ;
#4563=CARTESIAN_POINT ( 'NONE',  ( -105.6472514815422983, -266.3687386123619376, -319.2208520127341558 ) ) ;
#4564=CARTESIAN_POINT ( 'NONE',  ( -26.47192077230818796, -288.4178894023264093, -342.6606448618233003 ) ) ;
#4566=CARTESIAN_POINT ( 'NONE',  ( -66.47581498246137244, -284.3657095104144332, -341.3965489403619245 ) ) ;
#4567=CARTESIAN_POINT ( 'NONE',  ( 35.23409891286262763, -292.2928483653100784, -245.1886690202075272 ) ) ;
#4568=CARTESIAN_POINT ( 'NONE',  ( -17.22302613152774597, -281.9077621208018058, -196.8649999206666052 ) ) ;
#4569=CARTESIAN_POINT ( 'NONE',  ( -38.18140300432223455, -281.3570027617740266, -193.8588750487726884 ) ) ;
#4570=CARTESIAN_POINT ( 'NONE',  ( 35.13951695391511265, -281.5055051004177926, -279.4603423341849293 ) ) ;
#4571=CARTESIAN_POINT ( 'NONE',  ( 26.97827236433429121, -277.0346737862777786, -231.6867313962381445 ) ) ;
#4572=CARTESIAN_POINT ( 'NONE',  ( -89.60830321496932527, -297.3397075891438135, -213.7450823601406000 ) ) ;
#4573=CARTESIAN_POINT ( 'NONE',  ( -110.3132991166835808, -288.7750131857864062, -254.6451214292655436 ) ) ;
#4575=CARTESIAN_POINT ( 'NONE',  ( -106.6764805985710041, -271.6655836948855267, -246.2816927061899719 ) ) ;
#4577=CARTESIAN_POINT ( 'NONE',  ( -98.55372046247600792, -287.0512902252251024, -227.9781847445313474 ) ) ;
#4578=CARTESIAN_POINT ( 'NONE',  ( -69.38618270091909324, -296.5436682635711350, -340.0507645811265434 ) ) ;
#4579=CARTESIAN_POINT ( 'NONE',  ( -51.02886024927795461, -283.8829917290034928, -342.2219175641175184 ) ) ;
#4580=CARTESIAN_POINT ( 'NONE',  ( -51.28168796317569900, -276.2849532974807403, -345.8495074969753205 ) ) ;
#4581=CARTESIAN_POINT ( 'NONE',  ( -114.0866327045799977, -291.2643075570744031, -265.5105396513649225 ) ) ;
#4582=CARTESIAN_POINT ( 'NONE',  ( -111.7800741921122523, -282.8745649293283577, -255.9735814802576783 ) ) ;
#4584=CARTESIAN_POINT ( 'NONE',  ( 32.16504706785190137, -293.4598451725764789, -237.1531742276629871 ) ) ;
#4585=CARTESIAN_POINT ( 'NONE',  ( -94.96463191180620811, -290.2534627175618880, -315.2331318636522610 ) ) ;
#4588=CARTESIAN_POINT ( 'NONE',  ( 121.7894184752417601, 147.3656319919282964, -260.3019867207437983 ) ) ;
#4590=CARTESIAN_POINT ( 'NONE',  ( -76.38633874452972350, -285.0840267372630592, -335.9832136526091517 ) ) ;
#4591=CARTESIAN_POINT ( 'NONE',  ( -54.49178911615187104, -286.7666405000204009, -345.3538533559490702 ) ) ;
#4593=CARTESIAN_POINT ( 'NONE',  ( 36.01194568088035197, -280.4852213886582035, -271.3315130013310181 ) ) ;
#4594=CARTESIAN_POINT ( 'NONE',  ( -62.40312021176868029, -277.0360426768332331, -343.2025032670061933 ) ) ;
#4595=CARTESIAN_POINT ( 'NONE',  ( -94.50676637562121130, -281.2219457790112642, -222.0487110240886182 ) ) ;
#4596=CARTESIAN_POINT ( 'NONE',  ( 123.4377129911925266, 147.5673827398361482, -261.9833486453449041 ) ) ;
#4597=CARTESIAN_POINT ( 'NONE',  ( 35.04499807880887374, -280.4393464766956754, -294.9952549754937650 ) ) ;
#4598=CARTESIAN_POINT ( 'NONE',  ( -106.1031036191608194, -282.9550969145678891, -241.1815773895232837 ) ) ;
#4599=CARTESIAN_POINT ( 'NONE',  ( -3.987567352928275355, -300.2244201198217866, -194.3646069505561798 ) ) ;
#4600=CARTESIAN_POINT ( 'NONE',  ( -4.303226799851355366, -295.0968185298930280, -335.5399021057482400 ) ) ;
#4602=CARTESIAN_POINT ( 'NONE',  ( -67.99169109399944944, -290.3259492870271856, -203.5504249638108263 ) ) ;
#4603=CARTESIAN_POINT ( 'NONE',  ( -17.37636037328670824, -277.4524591733365355, -344.6221305986123298 ) ) ;
#4604=CARTESIAN_POINT ( 'NONE',  ( 25.27582940987185722, -275.0348354874549273, -232.7392820504886117 ) ) ;
#4605=CARTESIAN_POINT ( 'NONE',  ( 33.89201201114089201, -274.8360130969343800, -298.9163875505229271 ) ) ;
#4607=CARTESIAN_POINT ( 'NONE',  ( -80.44399200687146845, -271.4683023672242825, -208.9211940534819121 ) ) ;
#4610=CARTESIAN_POINT ( 'NONE',  ( 34.79206666094296452, -282.8045007752463107, -283.5061529161840213 ) ) ;
#4611=CARTESIAN_POINT ( 'NONE',  ( 25.89123344371115465, -283.8742959451880097, -312.4986324492521703 ) ) ;
#4612=CARTESIAN_POINT ( 'NONE',  ( -109.9750105505696638, -283.7861129506249540, -279.0622644067480564 ) ) ;
#4613=CARTESIAN_POINT ( 'NONE',  ( 24.64538066923214288, -274.5016016829282535, -310.5058020067859275 ) ) ;
#4614=CARTESIAN_POINT ( 'NONE',  ( 22.82676018172396581, -284.0109317930480870, -313.8641736651790666 ) ) ;
#4615=CARTESIAN_POINT ( 'NONE',  ( -46.00867426013731887, -275.6437788181847850, -343.5941307776746498 ) ) ;
#4617=CARTESIAN_POINT ( 'NONE',  ( -3.976223985848467368, -275.5826136997434332, -205.0709126687969501 ) ) ;
#4619=CARTESIAN_POINT ( 'NONE',  ( -41.01093377548058072, -280.8099413262089001, -193.5970834523247390 ) ) ;
#4623=CARTESIAN_POINT ( 'NONE',  ( -110.5342538430796253, -286.6639124639017382, -250.5893364286434633 ) ) ;
#4624=CARTESIAN_POINT ( 'NONE',  ( -28.88744741633575330, -294.1395400012453933, -343.0836092450228989 ) ) ;
#4625=CARTESIAN_POINT ( 'NONE',  ( -109.7723447150396510, -289.5725216538727409, -296.3475900868487543 ) ) ;
#4627=CARTESIAN_POINT ( 'NONE',  ( 11.82370490451610578, -284.9856325003853499, -214.9683122456135322 ) ) ;
#4628=CARTESIAN_POINT ( 'NONE',  ( 11.53889236592828027, -285.3204475261889570, -215.2829788251914067 ) ) ;
#4629=CARTESIAN_POINT ( 'NONE',  ( -109.4090960094531084, -289.0120973177457699, -253.4457738176095347 ) ) ;
#4630=CARTESIAN_POINT ( 'NONE',  ( -102.5983984975132586, -286.2114585151029473, -236.7650792044286163 ) ) ;
#4631=CARTESIAN_POINT ( 'NONE',  ( 36.75567406075547439, -273.7051210505691756, -282.2872240046474985 ) ) ;
#4632=CARTESIAN_POINT ( 'NONE',  ( -1.329459978771967643, -284.9215743562727425, -203.2078680525330867 ) ) ;
#4633=CARTESIAN_POINT ( 'NONE',  ( -34.17880835822248287, -300.0919018263072644, -195.3600309377237920 ) ) ;
#4634=CARTESIAN_POINT ( 'NONE',  ( 35.93817630864670321, -285.3369260564052183, -253.5680727324181589 ) ) ;
#4635=CARTESIAN_POINT ( 'NONE',  ( -4.251946925675381905, -281.4406959398218646, -205.0136029960060284 ) ) ;
#4636=CARTESIAN_POINT ( 'NONE',  ( -5.095886315687366164, -290.6288725320699768, -338.2739735961027350 ) ) ;
#4639=CARTESIAN_POINT ( 'NONE',  ( -73.88802776502943459, -297.4533385869179938, -336.5535102211179606 ) ) ;
#4640=CARTESIAN_POINT ( 'NONE',  ( -102.5381542272229751, -277.0462243174715127, -233.2879063699319317 ) ) ;
#4641=CARTESIAN_POINT ( 'NONE',  ( -33.53711398094534957, -291.2960718897893457, -193.6168416813030149 ) ) ;
#4642=CARTESIAN_POINT ( 'NONE',  ( -86.61949574754180503, -295.7533906512398403, -215.4235236385858059 ) ) ;
#4643=CARTESIAN_POINT ( 'NONE',  ( 20.07169716844475360, -279.5931799692712616, -224.4814352175958447 ) ) ;
#4644=CARTESIAN_POINT ( 'NONE',  ( -40.81819004538845519, -272.0880624479161725, -195.9516555355553749 ) ) ;
#4645=CARTESIAN_POINT ( 'NONE',  ( 26.65580675681370693, -294.3748127827618077, -234.1246795753736194 ) ) ;
#4646=CARTESIAN_POINT ( 'NONE',  ( -95.99890600148557951, -293.6948066931273615, -223.6242672951989618 ) ) ;
#4647=CARTESIAN_POINT ( 'NONE',  ( -107.7429233821329291, -294.6527196711982128, -299.9322141047771311 ) ) ;
#4648=CARTESIAN_POINT ( 'NONE',  ( -39.10706366233343090, -293.3138862350286331, -346.3272782651158082 ) ) ;
#4650=CARTESIAN_POINT ( 'NONE',  ( -94.55099831294803892, -291.3279414469306516, -316.6479532626935907 ) ) ;
#4652=CARTESIAN_POINT ( 'NONE',  ( -81.83533469017216078, -292.2313995384226928, -212.2201737899346199 ) ) ;
#4654=CARTESIAN_POINT ( 'NONE',  ( 0.03024653560056232010, -280.5775013590695721, -335.8110618514120347 ) ) ;
#4655=CARTESIAN_POINT ( 'NONE',  ( 35.20692541208019577, -293.6649332262791745, -278.9105385297491466 ) ) ;
#4656=CARTESIAN_POINT ( 'NONE',  ( 19.16016125881708021, -280.8395701745132556, -218.0491723122284498 ) ) ;
#4658=CARTESIAN_POINT ( 'NONE',  ( -97.15864897314560267, -283.5686332918953667, -318.8346656861278348 ) ) ;
#4659=CARTESIAN_POINT ( 'NONE',  ( -23.46969991109115838, -286.8743885574860428, -343.9504703888119366 ) ) ;
#4660=CARTESIAN_POINT ( 'NONE',  ( -98.56424538953238823, -282.1160091610662448, -312.4348571509264048 ) ) ;
#4662=CARTESIAN_POINT ( 'NONE',  ( 16.74545725553502606, -279.2844388542310412, -216.4605519834392169 ) ) ;
#4663=CARTESIAN_POINT ( 'NONE',  ( -40.78875968947717467, -284.9302148697245229, -193.6957519755633825 ) ) ;
#4665=CARTESIAN_POINT ( 'NONE',  ( 33.52401861852879961, -295.4223969751753884, -291.0097463781291367 ) ) ;
#4666=CARTESIAN_POINT ( 'NONE',  ( -23.03131561166794583, -278.2979531165901221, -345.4736618230061822 ) ) ;
#4667=CARTESIAN_POINT ( 'NONE',  ( -95.29238934966666363, -277.5940112745445276, -314.7886444228770415 ) ) ;
#4668=CARTESIAN_POINT ( 'NONE',  ( -112.8675802045441969, -290.5304660515217847, -285.4226547636037026 ) ) ;
#4669=CARTESIAN_POINT ( 'NONE',  ( 6.077178295763310700, -280.5484010394340544, -332.2645156247864406 ) ) ;
#4670=CARTESIAN_POINT ( 'NONE',  ( 35.85688529438362337, -292.5804076283258723, -268.0425969958330370 ) ) ;
#4671=CARTESIAN_POINT ( 'NONE',  ( -106.5398738202464983, -294.1727584096531132, -299.4199111992413691 ) ) ;
#4673=CARTESIAN_POINT ( 'NONE',  ( -26.20420625952874261, -294.4141798106948045, -342.5687676593620381 ) ) ;
#4675=CARTESIAN_POINT ( 'NONE',  ( -6.941161984400256557, -283.9809262143061233, -207.3071070584150277 ) ) ;
#4676=CARTESIAN_POINT ( 'NONE',  ( -104.0841914154499790, -272.2460806622759719, -232.1807672738869144 ) ) ;
#4677=CARTESIAN_POINT ( 'NONE',  ( 0.7734125911568857648, -278.6939772016694405, -204.8220396975919186 ) ) ;
#4678=CARTESIAN_POINT ( 'NONE',  ( -10.18477647504847283, -287.7143726996027340, -198.7798669876611086 ) ) ;
#4679=CARTESIAN_POINT ( 'NONE',  ( -0.9932859839907813848, -288.3889003757029741, -333.7264328488492993 ) ) ;
#4680=CARTESIAN_POINT ( 'NONE',  ( -98.21069622439456737, -279.4997387556539934, -311.9023392816845330 ) ) ;
#4681=CARTESIAN_POINT ( 'NONE',  ( -111.8855327853735702, -294.5221831127911400, -274.2423307797836856 ) ) ;
#4682=CARTESIAN_POINT ( 'NONE',  ( -111.1071850747128451, -298.2257558864490079, -277.0127101735137103 ) ) ;
#4683=CARTESIAN_POINT ( 'NONE',  ( -110.3004818743221733, -277.2360821265341428, -278.8204235032721385 ) ) ;
#4685=CARTESIAN_POINT ( 'NONE',  ( -62.83404288312284791, -297.3958719303138878, -197.7258321199578290 ) ) ;
#4686=CARTESIAN_POINT ( 'NONE',  ( -98.51867147455267570, -291.8925429663333944, -312.7944959491256327 ) ) ;
#4687=CARTESIAN_POINT ( 'NONE',  ( 1.380638594652329854, -296.1439354805377207, -335.9890152450253140 ) ) ;
#4688=CARTESIAN_POINT ( 'NONE',  ( -113.3111558597828576, -274.3094957117917829, -270.3834931753972910 ) ) ;
#4689=CARTESIAN_POINT ( 'NONE',  ( -58.71101569970753786, -289.9872201842382538, -340.3228271646576104 ) ) ;
#4692=CARTESIAN_POINT ( 'NONE',  ( -114.2640200941087016, -297.1770886592582315, -272.4752790926569901 ) ) ;
#4693=CARTESIAN_POINT ( 'NONE',  ( -113.0186961824049376, -288.6453862187887012, -274.0077254815403194 ) ) ;
#4694=CARTESIAN_POINT ( 'NONE',  ( -62.84204564026332918, -298.0623268394326715, -197.7286412917449638 ) ) ;
#4696=DIRECTION ( 'NONE',  ( -1.000000000000000000, -0.000000000000000000, -0.000000000000000000 ) ) ;
#4697=CARTESIAN_POINT ( 'NONE',  ( -41.70142007710229848, -290.6262233335039014, -346.5562439460481983 ) ) ;
#4698=CARTESIAN_POINT ( 'NONE',  ( 36.57525178469696669, -277.6233781216988064, -234.7283546768995564 ) ) ;
#4699=CARTESIAN_POINT ( 'NONE',  ( 30.63559147151739026, -280.4346265870901789, -234.2975993593122155 ) ) ;
#4700=CARTESIAN_POINT ( 'NONE',  ( -110.1551400786540711, -286.7751970328142193, -253.0364720606785909 ) ) ;
#4701=CARTESIAN_POINT ( 'NONE',  ( -3.732033264719329946, -285.0616457423262204, -201.7245701883663287 ) ) ;
#4702=CARTESIAN_POINT ( 'NONE',  ( -32.54879122782131162, -272.1125250118368513, -195.6685848506718060 ) ) ;
#4703=CARTESIAN_POINT ( 'NONE',  ( -40.86714032344767134, -275.9277501725102866, -195.9539622819045235 ) ) ;
#4704=CARTESIAN_POINT ( 'NONE',  ( -108.3326535388154923, -288.3388626676915578, -292.9281880220445942 ) ) ;
#4705=CARTESIAN_POINT ( 'NONE',  ( -59.28427648553832086, -279.1936555258983503, -342.8789007752742464 ) ) ;
#4707=CARTESIAN_POINT ( 'NONE',  ( 4.923154784574807152, -280.6413668813862046, -210.8406841869959862 ) ) ;
#4708=CARTESIAN_POINT ( 'NONE',  ( 35.62210993554892013, -280.8415650315028529, -265.8694491492755674 ) ) ;
#4709=CARTESIAN_POINT ( 'NONE',  ( -4.116277169682523329, -277.7039592856522745, -339.4954832554731752 ) ) ;
#4710=CARTESIAN_POINT ( 'NONE',  ( 31.67044634921600021, -279.9169872171020188, -236.9924942324666404 ) ) ;
#4711=CARTESIAN_POINT ( 'NONE',  ( 172.0061749996893354, 242.1526343824411072, -177.7416445279219772 ) ) ;
#4712=CARTESIAN_POINT ( 'NONE',  ( 38.50518149417412417, -276.6460587157657756, -282.5302153825796267 ) ) ;
#4714=CARTESIAN_POINT ( 'NONE',  ( -105.0032030312531504, -274.5327892572519772, -234.9675638856268165 ) ) ;
#4715=CARTESIAN_POINT ( 'NONE',  ( -6.941161984400275209, -279.1233781216987495, -333.4151289067050357 ) ) ;
#4719=CARTESIAN_POINT ( 'NONE',  ( 34.00508519049079581, -288.8531565856383736, -287.2093315194344427 ) ) ;
#4720=CARTESIAN_POINT ( 'NONE',  ( 33.89633579638270078, -288.9735314842162097, -243.9203114543053630 ) ) ;
#4721=CARTESIAN_POINT ( 'NONE',  ( -84.75744235378564895, -289.0744099093689101, -326.0664147626069962 ) ) ;
#4722=CARTESIAN_POINT ( 'NONE',  ( -20.99092746370978801, -285.7642222696639465, -195.1801420888355096 ) ) ;
#4723=CARTESIAN_POINT ( 'NONE',  ( -62.48528110653271739, -183.4704917803509829, -362.4204795493197366 ) ) ;
#4724=CARTESIAN_POINT ( 'NONE',  ( 34.42335972128890376, -280.1773038927441917, -287.6257651022099822 ) ) ;
#4725=CARTESIAN_POINT ( 'NONE',  ( 34.90707358132212335, -289.1905743615654956, -253.2481120857285077 ) ) ;
#4726=CARTESIAN_POINT ( 'NONE',  ( -4.535737291793926040, -281.0916447503937547, -336.3495757375241624 ) ) ;
#4727=CARTESIAN_POINT ( 'NONE',  ( -67.52402796698864051, -280.9628967905017589, -203.3379368807701155 ) ) ;
#4728=CARTESIAN_POINT ( 'NONE',  ( -45.90909642145814473, -277.6559237010195034, -342.9692679963890782 ) ) ;
#4729=CARTESIAN_POINT ( 'NONE',  ( -109.4967426273986746, -289.0189483437380318, -296.2411898321437889 ) ) ;
#4730=CARTESIAN_POINT ( 'NONE',  ( -112.0597234316401511, -285.1296096367069026, -288.3437432660147692 ) ) ;
#4731=CARTESIAN_POINT ( 'NONE',  ( -114.0909617899771575, -285.1208700617415275, -264.2593677967915369 ) ) ;
#4732=CARTESIAN_POINT ( 'NONE',  ( 26.85605756591158411, -282.1929873405071589, -305.1123469039780502 ) ) ;
#4735=CARTESIAN_POINT ( 'NONE',  ( -109.5965772592458620, -292.1194841406426121, -293.3257201945652355 ) ) ;
#4736=CARTESIAN_POINT ( 'NONE',  ( 20.02012098263473305, -291.5468765720261786, -219.7160324225135639 ) ) ;
#4737=CARTESIAN_POINT ( 'NONE',  ( 33.74044315437132013, -274.3790307910541628, -252.7333740770584711 ) ) ;
#4738=CARTESIAN_POINT ( 'NONE',  ( -103.0328220945177407, -295.3780743163102898, -310.3359760959696132 ) ) ;
#4739=CARTESIAN_POINT ( 'NONE',  ( -4.506929531580985859, -290.9727079686190905, -204.3729313823540679 ) ) ;
#4740=CARTESIAN_POINT ( 'NONE',  ( -50.67546114282041003, -293.4646461627337430, -343.1634862706560511 ) ) ;
#4741=CARTESIAN_POINT ( 'NONE',  ( -109.5669331250463614, -291.5858390791577222, -283.4242808501812760 ) ) ;
#4742=DIRECTION ( 'NONE',  ( 1.000000000000000000, 0.000000000000000000, 0.000000000000000000 ) ) ;
#4743=CARTESIAN_POINT ( 'NONE',  ( -106.9329693694158578, -292.1879274377781712, -298.3263802150158881 ) ) ;
#4744=CARTESIAN_POINT ( 'NONE',  ( -30.83008176695459923, -290.1339811200797953, -195.4255237265460039 ) ) ;
#4745=CARTESIAN_POINT ( 'NONE',  ( 37.05095200606859152, -295.4249422599753530, -260.4410809049220461 ) ) ;
#4746=CARTESIAN_POINT ( 'NONE',  ( -57.47052722810708758, -286.7272679176734869, -199.8935698004119104 ) ) ;
#4747=CARTESIAN_POINT ( 'NONE',  ( -19.69243258534993757, -296.8260355621781059, -343.4799579227356503 ) ) ;
#4748=CARTESIAN_POINT ( 'NONE',  ( -24.46599358326421481, -276.1954652938281924, -196.0610714254875973 ) ) ;
#4749=CARTESIAN_POINT ( 'NONE',  ( 22.32202329137529873, -274.9945508533119209, -318.4260988948511226 ) ) ;
#4750=CARTESIAN_POINT ( 'NONE',  ( 53.36098360292933762, -298.3578056523604687, -193.5345460460098650 ) ) ;
#4751=CARTESIAN_POINT ( 'NONE',  ( -5.865760172917629411, -274.8724399112180663, -337.3619337298343908 ) ) ;
#4752=CARTESIAN_POINT ( 'NONE',  ( 18.15231950314754528, -278.9359384421925370, -220.7453142062751965 ) ) ;
#4753=CARTESIAN_POINT ( 'NONE',  ( -110.7387727487133446, -273.7570339776519859, -270.3764257432318345 ) ) ;
#4754=CARTESIAN_POINT ( 'NONE',  ( -27.05771434395720831, -272.7550404801909281, -194.5925365816114549 ) ) ;
#4755=CARTESIAN_POINT ( 'NONE',  ( -105.5008819928261232, -297.6087568374248349, -298.1046008810332637 ) ) ;
#4757=CARTESIAN_POINT ( 'NONE',  ( -94.58404058921487945, -297.9969704448878360, -224.7988947476130477 ) ) ;
#4759=CARTESIAN_POINT ( 'NONE',  ( -3.815661055587151740, -286.6322703723892005, -337.8618123248742791 ) ) ;
#4760=CARTESIAN_POINT ( 'NONE',  ( -102.0294619080500524, -272.8471769016366579, -236.4212762380294635 ) ) ;
#4761=CARTESIAN_POINT ( 'NONE',  ( 25.54510566533832971, -286.9639087269663378, -225.9058560106946629 ) ) ;
#4762=CARTESIAN_POINT ( 'NONE',  ( -60.02509543646795720, -289.0050368228770026, -343.9220306246539280 ) ) ;
#4763=CARTESIAN_POINT ( 'NONE',  ( -109.6302365437836812, -298.2587740187327086, -291.6850719994691872 ) ) ;
#4764=CARTESIAN_POINT ( 'NONE',  ( 31.15825626278251548, -291.9474178855201671, -300.4905786151506391 ) ) ;
#4765=CARTESIAN_POINT ( 'NONE',  ( 36.32093819717986349, -281.0262658275285048, -292.4067044790296563 ) ) ;
#4767=CARTESIAN_POINT ( 'NONE',  ( -104.6370817574469498, -276.1139376130111600, -303.5881779673679830 ) ) ;
#4769=CARTESIAN_POINT ( 'NONE',  ( -37.28302428000554158, -287.8463238919713945, -343.7581687639628285 ) ) ;
#4772=CARTESIAN_POINT ( 'NONE',  ( -69.64177404394288828, -287.4772168803207251, -338.0494174040621260 ) ) ;
#4773=CARTESIAN_POINT ( 'NONE',  ( -50.11216171078302750, -299.4865958640592680, -197.6744223341751479 ) ) ;
#4774=CARTESIAN_POINT ( 'NONE',  ( 21.17060116043438356, -283.6441664382444969, -319.5029219026433225 ) ) ;
#4775=CARTESIAN_POINT ( 'NONE',  ( -100.0004653762155868, -271.2000396087570948, -228.0401388598519077 ) ) ;
#4776=CARTESIAN_POINT ( 'NONE',  ( -40.23435849278468623, -283.0895227110742098, -343.3037840127039431 ) ) ;
#4777=CARTESIAN_POINT ( 'NONE',  ( 9.849144460514617450, -276.1418520665376946, -213.8284904838072862 ) ) ;
#4778=ADVANCED_FACE ( 'NONE', ( #9230 ), #25439, .F. ) ;
#4779=CARTESIAN_POINT ( 'NONE',  ( 27.54323223260126241, -283.0500678251806903, -232.7453473655083087 ) ) ;
#4780=CARTESIAN_POINT ( 'NONE',  ( -56.93104289254733175, -272.7139623974682650, -199.6648252726962767 ) ) ;
#4782=ORIENTED_EDGE ( 'NONE', *, *, #13516, .T. ) ;
#4783=CARTESIAN_POINT ( 'NONE',  ( 203.6182477417019356, 295.8614695731350821, -54.00000000006011902 ) ) ;
#4784=CARTESIAN_POINT ( 'NONE',  ( 36.70474744800839062, -293.1201637223051080, -249.1914313631092739 ) ) ;
#4785=CARTESIAN_POINT ( 'NONE',  ( -111.9619450001418244, -286.4884964043978925, -273.7371169228075587 ) ) ;
#4787=CARTESIAN_POINT ( 'NONE',  ( -115.3288506153726871, -276.2666405000204009, -252.5284128619063608 ) ) ;
#4788=CARTESIAN_POINT ( 'NONE',  ( -114.2234999861203590, -277.7338498405199516, -271.5955770909419584 ) ) ;
#4789=CARTESIAN_POINT ( 'NONE',  ( -72.81966113325424317, -287.9139445196076394, -337.8127652717201954 ) ) ;
#4791=CARTESIAN_POINT ( 'NONE',  ( -93.07087735107516835, -285.3914876462631582, -318.5982219497129222 ) ) ;
#4793=CARTESIAN_POINT ( 'NONE',  ( -97.69925530789522838, -279.7220536453020259, -313.2193144267465073 ) ) ;
#4794=CARTESIAN_POINT ( 'NONE',  ( -71.45923539320028794, -284.9192038175204402, -338.7321650897167729 ) ) ;
#4795=CARTESIAN_POINT ( 'NONE',  ( -32.13275347443686059, -281.7799021204014593, -343.5731209595419386 ) ) ;
#4796=CARTESIAN_POINT ( 'NONE',  ( -7.218923341825066231, -282.4473899130564973, -201.6621481302328505 ) ) ;
#4797=CARTESIAN_POINT ( 'NONE',  ( 16.02550869841847714, -274.9506917812724396, -214.8548928671532110 ) ) ;
#4798=CARTESIAN_POINT ( 'NONE',  ( -17.35994470371500853, -276.6344976110535754, -344.7232686685538852 ) ) ;
#4799=CARTESIAN_POINT ( 'NONE',  ( -6.139478730825269182, -296.5590464803067334, -337.9461428114860837 ) ) ;
#4802=CARTESIAN_POINT ( 'NONE',  ( -69.03319148580604292, -293.6040565877264612, -339.1935961930356029 ) ) ;
#4803=CARTESIAN_POINT ( 'NONE',  ( 34.18287681988810078, -274.8625136281199275, -255.3928601204138999 ) ) ;
#4804=CARTESIAN_POINT ( 'NONE',  ( -85.03497123102626176, -298.4909342040351135, -210.3041083969167460 ) ) ;
#4805=CARTESIAN_POINT ( 'NONE',  ( 21.12757724937024051, -288.6818328797277786, -224.9814130557638521 ) ) ;
#4806=CARTESIAN_POINT ( 'NONE',  ( 36.03210093131030334, -294.8066932907680666, -249.3613887885495899 ) ) ;
#4807=CARTESIAN_POINT ( 'NONE',  ( 39.04396412927923876, -294.6847487297396810, -264.5957893989631771 ) ) ;
#4808=CARTESIAN_POINT ( 'NONE',  ( -110.4484133573006517, -292.3459322630665156, -286.4029862868962368 ) ) ;
#4809=CARTESIAN_POINT ( 'NONE',  ( -24.53829087852558999, -278.2157762149737437, -196.6311977641455542 ) ) ;
#4810=CARTESIAN_POINT ( 'NONE',  ( -69.16056666271923348, -281.5504392788729433, -203.0642091813285788 ) ) ;
#4811=CARTESIAN_POINT ( 'NONE',  ( -34.50117269507498463, -284.8772145006497567, -346.0726553238088741 ) ) ;
#4812=CARTESIAN_POINT ( 'NONE',  ( -19.72833028419634616, -285.2043201651664504, -199.1993636801954892 ) ) ;
#4813=CARTESIAN_POINT ( 'NONE',  ( 86.44575683232005758, 81.85753257257081827, -301.4767831277452501 ) ) ;
#4815=CARTESIAN_POINT ( 'NONE',  ( -109.4413297541693595, -284.3724205562562020, -258.7177366062745136 ) ) ;
#4817=CARTESIAN_POINT ( 'NONE',  ( 21.38222218702756194, -283.2986214375645773, -319.6865014955888569 ) ) ;
#4818=CARTESIAN_POINT ( 'NONE',  ( -64.58061434928194444, -274.0197913115372899, -202.5971427892014844 ) ) ;
#4819=CARTESIAN_POINT ( 'NONE',  ( -57.63588892406294661, -284.5908492520185291, -196.4402669667841508 ) ) ;
#4820=CARTESIAN_POINT ( 'NONE',  ( -45.26105567974459376, -280.8955505605646294, -193.9531714973741998 ) ) ;
#4821=CARTESIAN_POINT ( 'NONE',  ( -105.5644583403313419, -280.5172715435263058, -236.0620520223841936 ) ) ;
#4822=CARTESIAN_POINT ( 'NONE',  ( -6.279157895928174860, -281.1010252308510076, -200.0017785381950546 ) ) ;
#4823=CARTESIAN_POINT ( 'NONE',  ( -37.37352853689063181, -280.5523547857346784, -340.3611179825599606 ) ) ;
#4824=CARTESIAN_POINT ( 'NONE',  ( 65.82139847730509530, 47.41426247659997273, -318.9771648146296457 ) ) ;
#4826=CARTESIAN_POINT ( 'NONE',  ( -79.91857489696971584, -275.4753622649810723, -208.7576189306324466 ) ) ;
#4827=CARTESIAN_POINT ( 'NONE',  ( 179.3423712301919579, 254.3167496676224744, -166.5185575139265666 ) ) ;
#4828=CARTESIAN_POINT ( 'NONE',  ( -88.64315556899686044, -277.3486660267244588, -216.0678736075912525 ) ) ;
#4829=CARTESIAN_POINT ( 'NONE',  ( 16.75226959300215768, -294.5688739103903231, -216.9221133745738257 ) ) ;
#4830=CARTESIAN_POINT ( 'NONE',  ( -108.4000593501074690, -295.6739364221820097, -287.5779105873440358 ) ) ;
#4831=CARTESIAN_POINT ( 'NONE',  ( -99.15140905067138988, -290.6696191897650010, -224.5232583887171813 ) ) ;
#4834=CARTESIAN_POINT ( 'NONE',  ( -110.2431222966178979, -294.8365315187070337, -293.2957511565517734 ) ) ;
#4835=CARTESIAN_POINT ( 'NONE',  ( 35.91590325600594724, -286.0685564630210820, -279.2921851719104893 ) ) ;
#4836=CARTESIAN_POINT ( 'NONE',  ( 9.612090873140548553, -294.5660433463754089, -212.7948340075635372 ) ) ;
#4838=CARTESIAN_POINT ( 'NONE',  ( -99.43881027987846721, -285.3266107964624894, -309.7652917306182871 ) ) ;
#4840=CARTESIAN_POINT ( 'NONE',  ( -98.16919230591311418, -292.1203836765540700, -223.5121124017161378 ) ) ;
#4841=CARTESIAN_POINT ( 'NONE',  ( -8.464153608215625013, -283.1559737728903769, -337.4735292697905606 ) ) ;
#4842=CARTESIAN_POINT ( 'NONE',  ( -112.2091346281442412, -295.5516251887492558, -254.0865016796416285 ) ) ;
#4843=CARTESIAN_POINT ( 'NONE',  ( -75.57444452775595778, -290.3516462975356944, -337.0125701513002241 ) ) ;
#4844=CARTESIAN_POINT ( 'NONE',  ( -66.99752152933037053, -292.1660619823408069, -199.3677439231391020 ) ) ;
#4845=CARTESIAN_POINT ( 'NONE',  ( 33.70982118210871192, -287.4971128931756539, -253.5535546370061297 ) ) ;
#4848=CARTESIAN_POINT ( 'NONE',  ( -112.4252009086281134, -298.2788406506198271, -280.8821943108006849 ) ) ;
#4849=CARTESIAN_POINT ( 'NONE',  ( -31.93592802908120376, -296.8033309403293742, -193.8554441496146694 ) ) ;
#4850=CARTESIAN_POINT ( 'NONE',  ( 15.43724516592988927, -279.8795028648297603, -219.5167046605941437 ) ) ;
#4852=CARTESIAN_POINT ( 'NONE',  ( -18.55892191033718319, -273.7953345295165946, -195.6955810522516686 ) ) ;
#4853=CARTESIAN_POINT ( 'NONE',  ( -92.34965465860433653, -295.7267187377690902, -221.3220244783978217 ) ) ;
#4854=CARTESIAN_POINT ( 'NONE',  ( -4.498637119073520374, -278.4751869823304560, -336.9500054205054198 ) ) ;
#4855=CARTESIAN_POINT ( 'NONE',  ( 1.274900704134463769, -272.7134559620038203, -206.9606162493793988 ) ) ;
#4857=CARTESIAN_POINT ( 'NONE',  ( 10.56221645920129859, -295.5778869349519482, -325.9699777021423301 ) ) ;
#4858=CARTESIAN_POINT ( 'NONE',  ( -102.8145700360186083, -298.0788727304875465, -237.2703378846572093 ) ) ;
#4860=CARTESIAN_POINT ( 'NONE',  ( -1.068852149940670682, -296.1791649933183521, -337.3886918087338245 ) ) ;
#4861=CIRCLE ( 'NONE', #51675, 6.151811579824029153 ) ;
#4862=CARTESIAN_POINT ( 'NONE',  ( 50.92442080470556220, -297.1544086963463087, -195.2244517004290003 ) ) ;
#4863=CARTESIAN_POINT ( 'NONE',  ( -77.31782574601211877, -292.1516710513772068, -209.1581601406573441 ) ) ;
#4864=CARTESIAN_POINT ( 'NONE',  ( -97.84361190735582170, -288.5476566689508218, -312.2747138637416811 ) ) ;
#4866=CARTESIAN_POINT ( 'NONE',  ( 39.49247728902545163, -275.9828719430831825, -265.4374620945740162 ) ) ;
#4867=CARTESIAN_POINT ( 'NONE',  ( -81.96039047585614412, -297.7583462934829299, -212.4933984757655310 ) ) ;
#4869=CARTESIAN_POINT ( 'NONE',  ( -5.658979525416277134, -282.4466340785737088, -201.9899835612124548 ) ) ;
#4870=CARTESIAN_POINT ( 'NONE',  ( -6.414266453204220397, -279.1347559247186041, -200.3698526432170866 ) ) ;
#4871=CARTESIAN_POINT ( 'NONE',  ( -108.5651488163527745, -277.5320518653529120, -299.3530676111329853 ) ) ;
#4872=CARTESIAN_POINT ( 'NONE',  ( -37.55123024062151416, -282.2520423766524118, -343.5347520565074433 ) ) ;
#4873=CARTESIAN_POINT ( 'NONE',  ( 37.80882081822648644, -279.5109957560512726, -267.1614423308773780 ) ) ;
#4874=CARTESIAN_POINT ( 'NONE',  ( -1.419265025288412030, -273.1131209992068989, -206.1208858896487754 ) ) ;
#4875=CARTESIAN_POINT ( 'NONE',  ( -108.7132350886247849, -280.8517928231246970, -247.1495585002936650 ) ) ;
#4878=CARTESIAN_POINT ( 'NONE',  ( -113.5409431168329348, -270.9881429158849073, -267.5031164987000238 ) ) ;
#4879=CARTESIAN_POINT ( 'NONE',  ( 19.45216918942022488, -278.2340522687968019, -319.6196649199679314 ) ) ;
#4880=CARTESIAN_POINT ( 'NONE',  ( -67.84831361232535585, -271.6516253541363994, -201.8317462266525979 ) ) ;
#4882=CARTESIAN_POINT ( 'NONE',  ( -111.5880302844671235, -286.6545215665677233, -256.0599809794483122 ) ) ;
#4885=CARTESIAN_POINT ( 'NONE',  ( -13.57756048138342919, -286.7436221479175629, -341.5503320769163338 ) ) ;
#4886=DIRECTION ( 'NONE',  ( 3.961265963009670520E-15, 7.202301750926674102E-15, -1.000000000000000000 ) ) ;
#4887=CARTESIAN_POINT ( 'NONE',  ( -10.35822302490307578, -293.4869103911102002, -338.6181503568845983 ) ) ;
#4888=CARTESIAN_POINT ( 'NONE',  ( 33.45866640173591833, -285.4002933035421279, -247.9987146828482594 ) ) ;
#4890=CARTESIAN_POINT ( 'NONE',  ( -87.85530130619319777, -293.7581209928216595, -325.7991621610911466 ) ) ;
#4891=CARTESIAN_POINT ( 'NONE',  ( -32.33242597101487803, -284.5940918933791295, -194.2059996633515482 ) ) ;
#4892=CARTESIAN_POINT ( 'NONE',  ( -74.93061786766870114, -281.1431284043267169, -206.7924221029747116 ) ) ;
#4893=CARTESIAN_POINT ( 'NONE',  ( 37.72228080054952670, -288.9492813795278607, -285.6387973564200706 ) ) ;
#4894=CARTESIAN_POINT ( 'NONE',  ( 25.86636303626246303, -280.3545814169787036, -312.5359299505789750 ) ) ;
#4895=CARTESIAN_POINT ( 'NONE',  ( -96.55861513423624842, -289.9551460553725519, -313.0501912584443289 ) ) ;
#4896=CARTESIAN_POINT ( 'NONE',  ( -7.779263522804096276, -281.8725946465293646, -202.9571503172723794 ) ) ;
#4897=CARTESIAN_POINT ( 'NONE',  ( -38.36636668151981411, -280.8418215704745080, -197.1943884165333714 ) ) ;
#4898=CARTESIAN_POINT ( 'NONE',  ( 33.53423964131933843, -289.8640512299933221, -296.1062003288715232 ) ) ;
#4900=CARTESIAN_POINT ( 'NONE',  ( -29.83888329357132818, -274.1446523376640130, -193.7275239160685771 ) ) ;
#4901=CARTESIAN_POINT ( 'NONE',  ( -111.6119060365011677, -292.6284037242052136, -262.8922950790631035 ) ) ;
#4903=CARTESIAN_POINT ( 'NONE',  ( 13.79469577742117714, -295.1948066931273615, -206.1857440867352693 ) ) ;
#4905=CARTESIAN_POINT ( 'NONE',  ( -73.05090154096768629, -271.5802567210113239, -204.1603793793584032 ) ) ;
#4907=CARTESIAN_POINT ( 'NONE',  ( -108.6956756763882765, -294.6085409226148499, -297.2505245158820344 ) ) ;
#4908=CARTESIAN_POINT ( 'NONE',  ( -88.16405079995766414, -296.8251525760260279, -217.8016618235631086 ) ) ;
#4909=CARTESIAN_POINT ( 'NONE',  ( -56.22474751579643026, -290.8198502892797137, -341.6471563432843368 ) ) ;
#4910=CARTESIAN_POINT ( 'NONE',  ( -6.815334853809469351, -284.4060385047582713, -337.7999086390247498 ) ) ;
#4912=CARTESIAN_POINT ( 'NONE',  ( -105.9762053092477885, -291.5414491266811297, -304.0657165305063927 ) ) ;
#4913=CARTESIAN_POINT ( 'NONE',  ( -113.3217359044789845, -291.7490144751628236, -279.7604153408674392 ) ) ;
#4914=CARTESIAN_POINT ( 'NONE',  ( -52.51785430827889201, -287.8579096330275320, -196.9125986646392050 ) ) ;
#4915=CARTESIAN_POINT ( 'NONE',  ( -4.945919163748738079, -280.6337153502207116, -200.5076042538772185 ) ) ;
#4916=CARTESIAN_POINT ( 'NONE',  ( -96.29949634516779611, -293.9865766989832423, -317.6393263222292944 ) ) ;
#4917=CARTESIAN_POINT ( 'NONE',  ( -8.040852057305190925, -282.5122491631590265, -341.6248211671182275 ) ) ;
#4918=CARTESIAN_POINT ( 'NONE',  ( 0.05585840449479470560, -276.4159360852512464, -206.2191581809597949 ) ) ;
#4919=CARTESIAN_POINT ( 'NONE',  ( -102.0172624299486870, -280.6233781216988064, -301.5434626090942061 ) ) ;
#4920=CARTESIAN_POINT ( 'NONE',  ( 21.08624753894064696, -273.1299242581312683, -221.7797537773550403 ) ) ;
#4923=CARTESIAN_POINT ( 'NONE',  ( 2.742981955218880774, -280.1132504048805458, -209.2168044745507984 ) ) ;
#4925=CARTESIAN_POINT ( 'NONE',  ( -101.7547436198937589, -279.2093028552251326, -311.9183268072246165 ) ) ;
#4926=CARTESIAN_POINT ( 'NONE',  ( -65.77902170535318760, -284.7479032151845786, -199.0438594783251460 ) ) ;
#4927=CARTESIAN_POINT ( 'NONE',  ( -0.7752702841963073910, -294.3049853421233593, -205.9968502007601217 ) ) ;
#4928=CARTESIAN_POINT ( 'NONE',  ( 37.12823885938615831, -277.3570837300402445, -286.5673899319208999 ) ) ;
#4930=CARTESIAN_POINT ( 'NONE',  ( -73.72520433340224599, -274.8950556267691354, -203.0003704561559630 ) ) ;
#4932=CARTESIAN_POINT ( 'NONE',  ( 20.83563444569399437, -276.0051415752525941, -314.4564436579703965 ) ) ;
#4933=CARTESIAN_POINT ( 'NONE',  ( -93.55132711363044962, -297.8643276987417039, -319.7625983513416941 ) ) ;
#4935=CARTESIAN_POINT ( 'NONE',  ( -106.2767011911338670, -282.9348318859209144, -241.1076986055834652 ) ) ;
#4937=CARTESIAN_POINT ( 'NONE',  ( 35.43401436272014848, -292.9007211873821461, -245.1111015900268626 ) ) ;
#4938=CARTESIAN_POINT ( 'NONE',  ( 37.01909597755875581, -273.4810238765877557, -263.2894477876452015 ) ) ;
#4939=CARTESIAN_POINT ( 'NONE',  ( 30.97927332278542067, -289.5918030207013771, -304.2245906810972542 ) ) ;
#4940=CARTESIAN_POINT ( 'NONE',  ( -38.89038250136956520, -290.9525967321614530, -197.0683648794951637 ) ) ;
#4942=CARTESIAN_POINT ( 'NONE',  ( -81.57440894148207633, -290.0377729313602799, -208.0548280712945370 ) ) ;
#4943=CARTESIAN_POINT ( 'NONE',  ( -109.2004807792858116, -290.0477307534052898, -283.3381411446984544 ) ) ;
#4945=CARTESIAN_POINT ( 'NONE',  ( 34.78646382197024423, -288.9639754743878370, -296.5737237019787926 ) ) ;
#4946=CARTESIAN_POINT ( 'NONE',  ( -104.4631710304650198, -279.2715894534917993, -241.6070638233822194 ) ) ;
#4947=CARTESIAN_POINT ( 'NONE',  ( -95.35670707001334279, -294.7922099516945309, -320.5183854517390500 ) ) ;
#4948=CARTESIAN_POINT ( 'NONE',  ( -100.9169036468908303, -285.7758635820551376, -227.0061311238433177 ) ) ;
#4949=CARTESIAN_POINT ( 'NONE',  ( -23.79379967551184905, -286.5538590166527797, -194.5296199704773414 ) ) ;
#4950=CARTESIAN_POINT ( 'NONE',  ( 20.20025431565767349, -282.5189068736929698, -315.3167735296333376 ) ) ;
#4951=CARTESIAN_POINT ( 'NONE',  ( -99.96309284007092799, -248.1514199804641123, -334.2866369982713763 ) ) ;
#4952=CARTESIAN_POINT ( 'NONE',  ( -100.6449816371857224, -246.9771042453164682, -333.4387840234001601 ) ) ;
#4953=CARTESIAN_POINT ( 'NONE',  ( -108.6942105140528412, -263.8743016747102388, -305.4261820326353813 ) ) ;
#4954=CARTESIAN_POINT ( 'NONE',  ( 31.41000280236153230, -275.0836566985414038, -295.5243731600141359 ) ) ;
#4955=CARTESIAN_POINT ( 'NONE',  ( -7.393901917673681545, -275.5702496660196630, -337.2741619783982969 ) ) ;
#4956=CARTESIAN_POINT ( 'NONE',  ( -111.5610360496762183, -296.3161605688875966, -249.8907584823023740 ) ) ;
#4957=CARTESIAN_POINT ( 'NONE',  ( 197.9387763173789097, 281.7318850872235316, -110.5339443574438860 ) ) ;
#4959=CARTESIAN_POINT ( 'NONE',  ( 23.11797070549487287, -274.8672739589834464, -317.2644080136721527 ) ) ;
#4960=CARTESIAN_POINT ( 'NONE',  ( -51.78079317222831435, -275.6251783136739846, -197.7173767555002541 ) ) ;
#4962=CARTESIAN_POINT ( 'NONE',  ( -111.7376368498547379, -297.2552913091812457, -289.3367519162903250 ) ) ;
#4963=CARTESIAN_POINT ( 'NONE',  ( 14.13117871769071243, -288.7973272495085553, -322.2121660426234371 ) ) ;
#4965=CARTESIAN_POINT ( 'NONE',  ( -112.1462409552617885, -297.1341629097532859, -287.9804424136190164 ) ) ;
#4966=CARTESIAN_POINT ( 'NONE',  ( -113.3297600418439686, -297.1964372639040448, -258.2218421832878334 ) ) ;
#4967=CARTESIAN_POINT ( 'NONE',  ( 32.75077106834511653, -293.9891801096249537, -290.8032446466365286 ) ) ;
#4969=CARTESIAN_POINT ( 'NONE',  ( 17.86806103522776823, -278.1892442910119598, -321.9479037952636418 ) ) ;
#4970=CARTESIAN_POINT ( 'NONE',  ( 29.23647073066169710, -280.5579615726911697, -231.8011119115069505 ) ) ;
#4971=CARTESIAN_POINT ( 'NONE',  ( -26.97640279445920797, -277.8583732964011119, -342.8591804315925060 ) ) ;
#4972=CARTESIAN_POINT ( 'NONE',  ( -37.10728521600817231, -278.8093545905229007, -346.3603136168954961 ) ) ;
#4973=CARTESIAN_POINT ( 'NONE',  ( -81.60103170033016795, -275.6713841243881689, -331.3489722555592607 ) ) ;
#4974=CARTESIAN_POINT ( 'NONE',  ( -105.9043195660262313, -297.5429670248083198, -244.8564382559320620 ) ) ;
#4975=CARTESIAN_POINT ( 'NONE',  ( -107.2609801142003505, -295.4309342995090901, -247.2504198751506976 ) ) ;
#4977=CARTESIAN_POINT ( 'NONE',  ( -25.41132162454394106, -280.6926714256533728, -194.3532698887637196 ) ) ;
#4978=CARTESIAN_POINT ( 'NONE',  ( -103.1300894707911482, -278.2894091312853675, -302.1148870780011180 ) ) ;
#4979=CARTESIAN_POINT ( 'NONE',  ( -54.40801074653987257, -287.9516542541475133, -344.9945628488656553 ) ) ;
#4980=CARTESIAN_POINT ( 'NONE',  ( -29.33009274934805788, -300.1523752840889756, -195.1917187978136212 ) ) ;
#4983=CARTESIAN_POINT ( 'NONE',  ( -92.54027316206729381, -289.0655257662701842, -318.4547449679207034 ) ) ;
#4984=CARTESIAN_POINT ( 'NONE',  ( 17.83297878087867971, -279.0959254406582204, -221.0282808264427103 ) ) ;
#4985=CARTESIAN_POINT ( 'NONE',  ( -93.52843072218699660, -277.7970669226219229, -222.8188386279254019 ) ) ;
#4986=CARTESIAN_POINT ( 'NONE',  ( -10.47849546694213707, -280.7789102076216068, -339.8396795446543024 ) ) ;
#4987=CARTESIAN_POINT ( 'NONE',  ( -70.74467444915229919, -287.6118242585804978, -203.1961492263329205 ) ) ;
#4988=CARTESIAN_POINT ( 'NONE',  ( -69.93033913081247022, -280.8181370833739834, -204.5816185000254563 ) ) ;
#4991=CARTESIAN_POINT ( 'NONE',  ( -70.04914007322521741, -293.6214269492350581, -202.8687182185756797 ) ) ;
#4992=CARTESIAN_POINT ( 'NONE',  ( -106.6610099386179940, -276.3877442776427529, -301.6149065844991242 ) ) ;
#4994=CARTESIAN_POINT ( 'NONE',  ( 9.736015795006476736, -277.0351785203231429, -326.2859007832590805 ) ) ;
#4995=CARTESIAN_POINT ( 'NONE',  ( -104.1428859094904595, -286.0959762065048153, -304.9366175320544698 ) ) ;
#4998=CARTESIAN_POINT ( 'NONE',  ( -69.99422823214790412, -291.3989432542661007, -338.5158228649826242 ) ) ;
#5000=CARTESIAN_POINT ( 'NONE',  ( -31.34530361948588251, -292.9763882565214317, -345.1722658401024546 ) ) ;
#5001=CARTESIAN_POINT ( 'NONE',  ( 37.66507928011557027, -286.9590909606237688, -287.0987363539143189 ) ) ;
#5003=CARTESIAN_POINT ( 'NONE',  ( -63.46647306729474991, -272.3892828533277566, -201.6544512081398466 ) ) ;
#5004=CARTESIAN_POINT ( 'NONE',  ( 36.76941570174395935, -291.6254867809028610, -265.2545850194514401 ) ) ;
#5007=CARTESIAN_POINT ( 'NONE',  ( -113.3145806173120747, -289.1288763778699149, -262.6872617894036921 ) ) ;
#5008=CARTESIAN_POINT ( 'NONE',  ( -72.77583245151139124, -287.1747305923090039, -205.6098712105278423 ) ) ;
#5009=CARTESIAN_POINT ( 'NONE',  ( 13.58459175419786469, -284.9932857787292733, -213.8947004972047523 ) ) ;
#5011=CARTESIAN_POINT ( 'NONE',  ( -109.7762140521277985, -286.1482823676980729, -257.3049056694184742 ) ) ;
#5012=LINE ( 'NONE', #69401, #47218 ) ;
#5013=CARTESIAN_POINT ( 'NONE',  ( -102.3866143922282959, -285.8092800991270792, -236.8684194527228044 ) ) ;
#5014=CARTESIAN_POINT ( 'NONE',  ( -2.832048895173628011, -294.4858264621272497, -203.3579218688950618 ) ) ;
#5015=CARTESIAN_POINT ( 'NONE',  ( 36.18484919670623157, -273.8545614876391596, -287.8282825112267460 ) ) ;
#5016=CARTESIAN_POINT ( 'NONE',  ( 36.47439572649278006, -276.1600111458380979, -292.2463213957709058 ) ) ;
#5018=CARTESIAN_POINT ( 'NONE',  ( 21.11112761909973656, -290.9768259910583197, -222.4802122861924545 ) ) ;
#5019=CARTESIAN_POINT ( 'NONE',  ( -103.4115949214931049, -279.0689577831113297, -230.7129256192662012 ) ) ;
#5020=CARTESIAN_POINT ( 'NONE',  ( -109.1790465747947252, -298.2698734096895805, -290.6402318670120621 ) ) ;
#5023=CARTESIAN_POINT ( 'NONE',  ( -54.85775004620027318, -284.5071882890613324, -198.9331834819201674 ) ) ;
#5024=CARTESIAN_POINT ( 'NONE',  ( 32.47230984654849095, -279.1936863048373993, -242.8147828625224633 ) ) ;
#5026=CARTESIAN_POINT ( 'NONE',  ( 2.076564583637728223, -273.0497195135510538, -205.0242359065937592 ) ) ;
#5027=CARTESIAN_POINT ( 'NONE',  ( -92.80938918636424262, -277.2237864368000260, -317.9765371131321103 ) ) ;
#5028=CARTESIAN_POINT ( 'NONE',  ( 21.08463185388143657, -295.6985930922944021, -315.2936044259757296 ) ) ;
#5030=CARTESIAN_POINT ( 'NONE',  ( 38.36049495791547059, -280.6276452433605755, -282.7178377671999101 ) ) ;
#5031=CARTESIAN_POINT ( 'NONE',  ( 6.212465513629102709, -295.3860070676503824, -329.3008315412002958 ) ) ;
#5032=CARTESIAN_POINT ( 'NONE',  ( -13.91701166505555598, -296.0695788362795611, -343.1936810450267217 ) ) ;
#5033=CARTESIAN_POINT ( 'NONE',  ( -65.57075502926024058, -297.5057496763832319, -203.0400925603047426 ) ) ;
#5034=CARTESIAN_POINT ( 'NONE',  ( -109.6876677991897111, -292.8066095137401703, -250.5858401657527565 ) ) ;
#5035=CARTESIAN_POINT ( 'NONE',  ( -83.27758010909099085, -285.6092075321863035, -208.4974189148646246 ) ) ;
#5036=CARTESIAN_POINT ( 'NONE',  ( 22.52719625648783008, -274.3221202761614563, -316.8151213583173558 ) ) ;
#5037=CARTESIAN_POINT ( 'NONE',  ( 36.78383620576741464, -287.6472096046332467, -291.2518487455981244 ) ) ;
#5038=CARTESIAN_POINT ( 'NONE',  ( -46.68682590685827449, -281.9129743228164671, -196.2513484276414033 ) ) ;
#5039=CARTESIAN_POINT ( 'NONE',  ( 23.69900906503054117, -287.1708816242754096, -310.8493154275352595 ) ) ;
#5040=CARTESIAN_POINT ( 'NONE',  ( -110.3226133027325488, -288.3293463810759363, -287.7016012181065321 ) ) ;
#5041=CARTESIAN_POINT ( 'NONE',  ( 202.9739649223127742, 291.4636489454787807, -68.19743562414970484 ) ) ;
#5042=CARTESIAN_POINT ( 'NONE',  ( 27.71579033283434867, -286.6071144906486552, -237.0003213354131617 ) ) ;
#5044=CARTESIAN_POINT ( 'NONE',  ( 36.25654271108132320, -282.7700688847044148, -292.3642315058255008 ) ) ;
#5045=CARTESIAN_POINT ( 'NONE',  ( -81.78437819734608638, -290.5217153100768428, -207.7698360146215748 ) ) ;
#5046=CARTESIAN_POINT ( 'NONE',  ( -38.18174308455428445, -281.6419110099115528, -194.1657457726626603 ) ) ;
#5047=CARTESIAN_POINT ( 'NONE',  ( 31.56994647985871794, -282.4368314243427562, -237.0055265298853442 ) ) ;
#5048=CARTESIAN_POINT ( 'NONE',  ( 18.49298438396720101, -282.0537006252001220, -317.4069823893198645 ) ) ;
#5049=CARTESIAN_POINT ( 'NONE',  ( 8.534723961188817043, -276.6807212584855620, -211.0285438057990461 ) ) ;
#5050=CARTESIAN_POINT ( 'NONE',  ( -88.60543184964716090, -295.7476945571318652, -327.8872069434855234 ) ) ;
#5051=CARTESIAN_POINT ( 'NONE',  ( -109.6967354547859657, -288.8096750788182590, -251.9626610498688137 ) ) ;
#5052=CARTESIAN_POINT ( 'NONE',  ( -41.87377477762861133, -296.9140259600816307, -197.1922286007973071 ) ) ;
#5055=CARTESIAN_POINT ( 'NONE',  ( -110.3879110723479755, -286.2868295445725266, -284.6986654427787471 ) ) ;
#5056=VECTOR ( 'NONE', #90212, 1000.000000000000000 ) ;
#5057=CARTESIAN_POINT ( 'NONE',  ( 31.90093501509288387, -294.2061152915784419, -237.2688259575994323 ) ) ;
#5058=CARTESIAN_POINT ( 'NONE',  ( 20.26641750026905697, -282.8369874063569682, -315.3633118388252115 ) ) ;
#5059=EDGE_CURVE ( 'NONE', #3540, #71727, #67204, .T. ) ;
#5060=CARTESIAN_POINT ( 'NONE',  ( 33.50105024918833863, -274.2322092032831051, -240.6581716900169567 ) ) ;
#5061=CARTESIAN_POINT ( 'NONE',  ( -114.2880357200276222, -291.1926095281505695, -271.2358884801321892 ) ) ;
#5062=CARTESIAN_POINT ( 'NONE',  ( -64.08860717743114321, -283.8465434078051999, -199.4605909208435151 ) ) ;
#5063=CARTESIAN_POINT ( 'NONE',  ( -13.87693914222193925, -292.6816548335221455, -196.9897498673465464 ) ) ;
#5065=CARTESIAN_POINT ( 'NONE',  ( 32.33507116531379921, -288.1768837280231423, -292.3751480622312897 ) ) ;
#5069=CARTESIAN_POINT ( 'NONE',  ( 84.55120471034096852, 81.53809721804566379, -298.7488921200802565 ) ) ;
#5070=CARTESIAN_POINT ( 'NONE',  ( 1.755669219107143464, -284.0592657388145312, -335.8905271248909230 ) ) ;
#5071=CARTESIAN_POINT ( 'NONE',  ( -114.2704648735229114, -288.0523547857346784, -270.3284710469133074 ) ) ;
#5073=CARTESIAN_POINT ( 'NONE',  ( 10.09830747003844920, -281.3006949694444643, -326.3176821264667069 ) ) ;
#5074=CARTESIAN_POINT ( 'NONE',  ( 19.85864627916476977, -275.9185262159213039, -321.8965172615079950 ) ) ;
#5075=CARTESIAN_POINT ( 'NONE',  ( -7.285914942196468402, -282.4473899109673312, -201.8147896459126116 ) ) ;
#5076=CARTESIAN_POINT ( 'NONE',  ( 27.32813335771293239, -24.61695715926212102, -343.0477418883668861 ) ) ;
#5077=CARTESIAN_POINT ( 'NONE',  ( 35.90857445423406347, -280.4039265822380571, -292.2916365071041582 ) ) ;
#5078=CARTESIAN_POINT ( 'NONE',  ( -84.67175412479804208, -283.4168336077982531, -212.5729866804885546 ) ) ;
#5080=CARTESIAN_POINT ( 'NONE',  ( -67.79224647856602814, -299.4182591044454966, -200.6865393352724993 ) ) ;
#5081=CARTESIAN_POINT ( 'NONE',  ( 12.40135767224208685, -294.8293791304913043, -323.9432353398989335 ) ) ;
#5083=CARTESIAN_POINT ( 'NONE',  ( -86.24477230005112460, -290.0418852153470084, -215.4316006113672586 ) ) ;
#5084=CARTESIAN_POINT ( 'NONE',  ( 31.76732283218936104, -276.6384922139824880, -304.2056527103570147 ) ) ;
#5085=CARTESIAN_POINT ( 'NONE',  ( -43.48212421531537331, -273.9725701068415447, -197.5691177544540835 ) ) ;
#5086=CARTESIAN_POINT ( 'NONE',  ( -27.02443708261399280, -273.1005857086767037, -194.3141744618107225 ) ) ;
#5088=CARTESIAN_POINT ( 'NONE',  ( 30.22679961042809538, -273.1219261130304972, -237.6930814542139387 ) ) ;
#5092=CARTESIAN_POINT ( 'NONE',  ( 35.87533242312211001, -282.6800807273444889, -274.0342933361034738 ) ) ;
#5093=CARTESIAN_POINT ( 'NONE',  ( 33.37305974970083611, -282.9533825498997430, -242.4076021657018885 ) ) ;
#5094=CARTESIAN_POINT ( 'NONE',  ( -84.93441606973981095, -283.0780242595014329, -325.8482881856795643 ) ) ;
#5095=CARTESIAN_POINT ( 'NONE',  ( -35.34851826131681918, -272.4774188881562509, -196.5753937415116468 ) ) ;
#5096=CARTESIAN_POINT ( 'NONE',  ( 33.14203194492596793, -283.1064974253362720, -246.8988552184602270 ) ) ;
#5097=CARTESIAN_POINT ( 'NONE',  ( 29.72499716802074943, -273.6226756817299020, -239.6963876090953818 ) ) ;
#5099=CARTESIAN_POINT ( 'NONE',  ( 33.80587072756687661, -276.3996271837275458, -252.6905425564350764 ) ) ;
#5101=CARTESIAN_POINT ( 'NONE',  ( -20.15226036016875000, -277.6396767212351619, -345.3068580607388185 ) ) ;
#5106=CARTESIAN_POINT ( 'NONE',  ( -86.95920298751730115, -287.2309480093535967, -213.0342522295029539 ) ) ;
#5107=CARTESIAN_POINT ( 'NONE',  ( -94.90681123830276533, -295.1140213192787201, -315.5148521626750835 ) ) ;
#5108=CARTESIAN_POINT ( 'NONE',  ( -17.75830013185584022, -288.1545815999714364, -344.7237647272082768 ) ) ;
#5109=CARTESIAN_POINT ( 'NONE',  ( -14.22856941916255558, -284.5957515971525140, -199.9955003492453329 ) ) ;
#5110=CARTESIAN_POINT ( 'NONE',  ( -65.30040432951437879, -284.2542696943920646, -202.2357010858243598 ) ) ;
#5111=CARTESIAN_POINT ( 'NONE',  ( -83.19132075283120287, -287.9299288940537735, -328.4626351696686015 ) ) ;
#5112=CARTESIAN_POINT ( 'NONE',  ( -78.58716304388681806, -284.8265352353776620, -331.0730796778912577 ) ) ;
#5113=CARTESIAN_POINT ( 'NONE',  ( -38.53925083100407534, -275.0670126289074915, -345.3515608738567835 ) ) ;
#5114=CARTESIAN_POINT ( 'NONE',  ( 1.135500732134293589, -284.9566924188076200, -204.5740170980117796 ) ) ;
#5115=CARTESIAN_POINT ( 'NONE',  ( -108.9124582445111997, -298.8435117785385842, -247.7694212526806723 ) ) ;
#5116=CARTESIAN_POINT ( 'NONE',  ( 32.17388447191516576, -285.1782093035108687, -241.6311128308203706 ) ) ;
#5118=CARTESIAN_POINT ( 'NONE',  ( 34.79680009934898521, -282.3273694958396050, -257.7339554567607820 ) ) ;
#5119=CARTESIAN_POINT ( 'NONE',  ( -20.87267618207762609, -290.8415605568310980, -343.7547885268265873 ) ) ;
#5122=CARTESIAN_POINT ( 'NONE',  ( -41.83501847219821457, -297.0283678103869534, -345.8388161005366896 ) ) ;
#5123=CARTESIAN_POINT ( 'NONE',  ( -7.172173674521296505, -278.4477156150321662, -201.6826648416823673 ) ) ;
#5124=CARTESIAN_POINT ( 'NONE',  ( -8.562192552985097294, -291.6165615031683842, -199.1157759289823730 ) ) ;
#5125=CARTESIAN_POINT ( 'NONE',  ( -104.6747840226607451, -294.5480159960924311, -300.6969782868713423 ) ) ;
#5126=CARTESIAN_POINT ( 'NONE',  ( 21.39400427248041225, -280.8533649351057875, -314.5561145920430022 ) ) ;
#5127=CARTESIAN_POINT ( 'NONE',  ( 20.99903835387845419, -272.9918385989889771, -224.1057428699021443 ) ) ;
#5128=CARTESIAN_POINT ( 'NONE',  ( 36.02583457602933237, -294.8005654733542542, -265.2655767428273634 ) ) ;
#5129=CARTESIAN_POINT ( 'NONE',  ( -95.95921662488163406, -292.4090924074130839, -317.1477375740089997 ) ) ;
#5130=CARTESIAN_POINT ( 'NONE',  ( -107.1310066386831892, -295.4308000253812452, -239.3734549974685422 ) ) ;
#5131=CARTESIAN_POINT ( 'NONE',  ( -36.36852897070759383, -290.3040614007007889, -194.3678186611271315 ) ) ;
#5132=CARTESIAN_POINT ( 'NONE',  ( -104.0984007623582954, -292.3920682971040605, -239.3947194858239698 ) ) ;
#5134=CARTESIAN_POINT ( 'NONE',  ( -49.72609649922945607, -292.6931247937685612, -198.2040023265234083 ) ) ;
#5136=CARTESIAN_POINT ( 'NONE',  ( -86.27125971562368534, -292.5959736771948201, -211.3523733338774946 ) ) ;
#5137=CARTESIAN_POINT ( 'NONE',  ( 33.04203922870224375, -279.9204885338987765, -297.2783250247895808 ) ) ;
#5138=CARTESIAN_POINT ( 'NONE',  ( -32.15728590108069085, -292.1193325364559428, -197.5328273110813484 ) ) ;
#5140=CARTESIAN_POINT ( 'NONE',  ( 39.61980569469341162, -281.5825985165997167, -272.7955833224256708 ) ) ;
#5141=CARTESIAN_POINT ( 'NONE',  ( -99.77381981583235415, -283.6206010088851599, -315.4832449321209538 ) ) ;
#5142=CARTESIAN_POINT ( 'NONE',  ( -91.94756060828976274, -287.8330834983093496, -321.6054472438466405 ) ) ;
#5143=CARTESIAN_POINT ( 'NONE',  ( -79.09052343481252478, -281.7615372537368330, -331.7443504719050793 ) ) ;
#5145=CARTESIAN_POINT ( 'NONE',  ( -81.81889464704876502, -277.9382048940400409, -208.3571913424385116 ) ) ;
#5147=CARTESIAN_POINT ( 'NONE',  ( 5.020432208683907049, -285.5302226169452524, -206.3686620744306310 ) ) ;
#5148=CARTESIAN_POINT ( 'NONE',  ( 121.3395553409046670, -299.5541904835127980, -192.6222259952039622 ) ) ;
#5149=CARTESIAN_POINT ( 'NONE',  ( 27.87446622108598859, -295.6190312693804003, -305.0144347577275425 ) ) ;
#5150=CARTESIAN_POINT ( 'NONE',  ( -17.49333229435270098, -278.2261936918599190, -344.1489800311915701 ) ) ;
#5151=CARTESIAN_POINT ( 'NONE',  ( -64.34490735153218566, -277.0810877185979848, -338.2595982287882634 ) ) ;
#5152=CARTESIAN_POINT ( 'NONE',  ( -86.51466323652709889, -291.5577450825049937, -211.0380268287154024 ) ) ;
#5154=CARTESIAN_POINT ( 'NONE',  ( -96.92429515610150759, -281.9993398261785273, -316.8286181507845072 ) ) ;
#5156=CARTESIAN_POINT ( 'NONE',  ( 25.99015165447522691, -293.1138321019154773, -307.1372651085534926 ) ) ;
#5157=CARTESIAN_POINT ( 'NONE',  ( -109.6859245714938282, -294.8085908961669475, -250.3878057391564198 ) ) ;
#5161=CARTESIAN_POINT ( 'NONE',  ( 27.54406242065528687, -292.6034922699741969, -236.7779933522577664 ) ) ;
#5163=CARTESIAN_POINT ( 'NONE',  ( -6.941161984400256557, -289.9809262143061233, -207.3071070584150277 ) ) ;
#5164=CARTESIAN_POINT ( 'NONE',  ( -86.25463878613970792, -294.7707406654784563, -329.5248285162815023 ) ) ;
#5165=CARTESIAN_POINT ( 'NONE',  ( 21.03439454779123352, -279.0319637508834489, -222.0647718033168587 ) ) ;
#5166=CARTESIAN_POINT ( 'NONE',  ( -30.94190509126000066, -287.4465713232191320, -194.1091984313555656 ) ) ;
#5167=CARTESIAN_POINT ( 'NONE',  ( -17.16983973862676649, -286.1530880547942388, -200.1506183683458744 ) ) ;
#5168=CARTESIAN_POINT ( 'NONE',  ( -109.4391165252961997, -279.8729500919551469, -285.6146521058996086 ) ) ;
#5169=CARTESIAN_POINT ( 'NONE',  ( -109.1927484744432348, -294.3107287378887804, -290.5916309758698048 ) ) ;
#5170=CARTESIAN_POINT ( 'NONE',  ( -109.2786872212679015, -298.0850999727042563, -287.8226540892346179 ) ) ;
#5172=CARTESIAN_POINT ( 'NONE',  ( -110.5536381880899768, -277.4154249027404830, -265.1512591097055633 ) ) ;
#5175=CARTESIAN_POINT ( 'NONE',  ( -112.5789292484276984, -296.4232784899679132, -254.0176057555253522 ) ) ;
#5176=CARTESIAN_POINT ( 'NONE',  ( -73.02812715167979718, -291.4491800446547245, -335.6894665437833964 ) ) ;
#5178=CARTESIAN_POINT ( 'NONE',  ( -53.42289092708005427, -289.9153492663852489, -341.6723230650061964 ) ) ;
#5182=CARTESIAN_POINT ( 'NONE',  ( 11.33411921951718426, -281.4554532092836894, -329.7888444128520291 ) ) ;
#5183=CARTESIAN_POINT ( 'NONE',  ( -101.5385901050513553, -296.6450866686284940, -312.7902762043616463 ) ) ;
#5184=CARTESIAN_POINT ( 'NONE',  ( -89.91155455344491543, -289.4594214597105974, -215.7290396917294402 ) ) ;
#5185=CARTESIAN_POINT ( 'NONE',  ( -102.3008286208124247, -297.4269585560355722, -229.0566882328157874 ) ) ;
#5186=CARTESIAN_POINT ( 'NONE',  ( 16.17752346111596751, -294.5992251257119960, -320.0378750546560696 ) ) ;
#5190=CARTESIAN_POINT ( 'NONE',  ( -59.80454023100995187, -290.8581414735180601, -343.2866180892807506 ) ) ;
#5191=CARTESIAN_POINT ( 'NONE',  ( 36.60358173371528068, -278.4805209788416391, -305.9350535429201159 ) ) ;
#5193=CARTESIAN_POINT ( 'NONE',  ( -6.263947264179056340, -279.7984094211952879, -200.0084954448707890 ) ) ;
#5194=CARTESIAN_POINT ( 'NONE',  ( -92.89900469587266230, -287.2533497265698088, -220.1509817255634118 ) ) ;
#5195=CARTESIAN_POINT ( 'NONE',  ( 1.239958049647971627, -285.1315202942427618, -204.3908957128678878 ) ) ;
#5196=CARTESIAN_POINT ( 'NONE',  ( 18.67441364952511407, -272.8596833560802679, -220.6635065063786669 ) ) ;
#5197=CARTESIAN_POINT ( 'NONE',  ( -59.93553525168671570, -275.6774021192776445, -199.3787818580472617 ) ) ;
#5198=CARTESIAN_POINT ( 'NONE',  ( -107.9291627250842964, -288.9398651247442444, -246.7237678453780063 ) ) ;
#5199=CARTESIAN_POINT ( 'NONE',  ( -110.9691125764410344, -280.1847479181629410, -288.2846260749583394 ) ) ;
#5201=CARTESIAN_POINT ( 'NONE',  ( -72.12970831731853139, -279.5783575795214233, -206.1832831310665313 ) ) ;
#5202=CARTESIAN_POINT ( 'NONE',  ( 35.80471126089338441, -280.9134106719703254, -271.3233667817196988 ) ) ;
#5203=CARTESIAN_POINT ( 'NONE',  ( 39.24476117293337296, -276.5701015933856866, -265.4458315290269184 ) ) ;
#5204=CARTESIAN_POINT ( 'NONE',  ( -92.77575336046501775, -278.0743631382828767, -217.4168829144651056 ) ) ;
#5205=CARTESIAN_POINT ( 'NONE',  ( 83.01528650091917427, 82.86587161941417889, -299.6803353214908725 ) ) ;
#5206=CARTESIAN_POINT ( 'NONE',  ( -110.8154329800676834, -273.7754314059740182, -247.9435182257268480 ) ) ;
#5208=CARTESIAN_POINT ( 'NONE',  ( -54.48078351602919156, -299.2613780133917203, -195.8973139439567888 ) ) ;
#5209=CARTESIAN_POINT ( 'NONE',  ( 10.64812456238590066, -290.9090924074130839, -330.4860931364851808 ) ) ;
#5212=CARTESIAN_POINT ( 'NONE',  ( 35.96440432506301477, -288.6405545456452728, -271.0252885460425887 ) ) ;
#5213=CARTESIAN_POINT ( 'NONE',  ( 35.81498924262982086, -289.5737196124663342, -290.9532980691903958 ) ) ;
#5215=CARTESIAN_POINT ( 'NONE',  ( -107.4907741942367352, -290.1729894693338565, -249.7497225756217745 ) ) ;
#5216=CARTESIAN_POINT ( 'NONE',  ( -111.6601301425914130, -284.3115295270666252, -250.2537107587252194 ) ) ;
#5217=CARTESIAN_POINT ( 'NONE',  ( -38.34447141573473772, -278.4392501149724239, -196.5553919712435516 ) ) ;
#5218=CARTESIAN_POINT ( 'NONE',  ( -75.37291989161539618, -287.3996389462576531, -206.6077509852390506 ) ) ;
#5219=CARTESIAN_POINT ( 'NONE',  ( 24.70382933162989758, -280.5780566252981885, -310.2174366137197694 ) ) ;
#5220=CARTESIAN_POINT ( 'NONE',  ( -109.0918435712439560, -280.0765010432311897, -254.3924322468265586 ) ) ;
#5222=CARTESIAN_POINT ( 'NONE',  ( -13.75960945927488410, -277.2301571350907352, -339.5653938045198856 ) ) ;
#5223=CARTESIAN_POINT ( 'NONE',  ( -84.93007324650470480, -288.4866295489613890, -330.4567619164132566 ) ) ;
#5224=CARTESIAN_POINT ( 'NONE',  ( -99.65151941333596142, -284.7565312445059362, -315.4127301472503859 ) ) ;
#5225=CARTESIAN_POINT ( 'NONE',  ( -90.39116480040159729, -284.2710423361637027, -326.1592125277091441 ) ) ;
#5226=CARTESIAN_POINT ( 'NONE',  ( 1.103112464788249314, -282.6903604730115376, -332.4765417471646174 ) ) ;
#5229=CARTESIAN_POINT ( 'NONE',  ( -94.74088923696332643, -293.0913761484256383, -220.8878821829949288 ) ) ;
#5230=CARTESIAN_POINT ( 'NONE',  ( -39.18292794993724470, -290.7143634581076981, -193.8634737358342761 ) ) ;
#5232=CARTESIAN_POINT ( 'NONE',  ( 17.46960225621667462, -273.9184208313080262, -221.7150878113808972 ) ) ;
#5233=CARTESIAN_POINT ( 'NONE',  ( -53.27623570813805998, -294.5997837917406059, -345.6445963459857467 ) ) ;
#5234=CARTESIAN_POINT ( 'NONE',  ( -82.13527866676525946, -289.9088187613551213, -211.7795256885372908 ) ) ;
#5235=CARTESIAN_POINT ( 'NONE',  ( -72.62714917692127869, -293.7658967764913882, -335.4364132261795248 ) ) ;
#5236=CARTESIAN_POINT ( 'NONE',  ( -53.48098859572185404, -290.4689226899012624, -341.9617735058484413 ) ) ;
#5239=CARTESIAN_POINT ( 'NONE',  ( -109.3201032708799545, -292.8236813696574359, -249.2871973460374591 ) ) ;
#5240=CARTESIAN_POINT ( 'NONE',  ( 29.28595432435684387, -291.0908401502043716, -235.4526725880037077 ) ) ;
#5241=CARTESIAN_POINT ( 'NONE',  ( -9.761006749027520968, -296.6922007399874133, -340.1605706291933870 ) ) ;
#5242=CARTESIAN_POINT ( 'NONE',  ( -38.64106608655507102, -286.9767521562553725, -197.1248289421772881 ) ) ;
#5243=CARTESIAN_POINT ( 'NONE',  ( -41.81048221307512591, -297.1083613095757414, -345.4459798781037421 ) ) ;
#5244=CARTESIAN_POINT ( 'NONE',  ( 37.98056521063064395, -277.5777847643498717, -273.9401515419625071 ) ) ;
#5246=CARTESIAN_POINT ( 'NONE',  ( -87.34940106855336239, -296.5728717160762926, -211.9524152496438489 ) ) ;
#5247=CARTESIAN_POINT ( 'NONE',  ( 32.20636937398665367, -274.1265022785975702, -295.8286906556134568 ) ) ;
#5248=CARTESIAN_POINT ( 'NONE',  ( -24.60645761907724349, -278.2957697506427621, -197.0185805737351359 ) ) ;
#5249=CARTESIAN_POINT ( 'NONE',  ( -36.49292348757258964, -299.3781713783291707, -196.8677687253267550 ) ) ;
#5250=CARTESIAN_POINT ( 'NONE',  ( -5.344347276814142234, -273.0397253587576074, -200.9725331469751666 ) ) ;
#5251=CARTESIAN_POINT ( 'NONE',  ( -45.13523733884863276, -296.5779169706398761, -343.5873780670190172 ) ) ;
#5253=CARTESIAN_POINT ( 'NONE',  ( -104.0797307080208327, -296.9505903062203060, -300.4621927159616348 ) ) ;
#5255=CARTESIAN_POINT ( 'NONE',  ( -90.45744271053995078, -287.8193310567069148, -323.8866247585355609 ) ) ;
#5256=CARTESIAN_POINT ( 'NONE',  ( -37.14961190020886761, -298.0546309613013136, -197.3582692470340874 ) ) ;
#5257=CARTESIAN_POINT ( 'NONE',  ( 33.85942663172103551, -287.1780478192079613, -240.9063071331173660 ) ) ;
#5258=CARTESIAN_POINT ( 'NONE',  ( -71.90078118066590207, -289.1632299533132482, -339.1463940846297760 ) ) ;
#5259=CARTESIAN_POINT ( 'NONE',  ( -112.0190556993653246, -298.3982976316639224, -280.8269497424009273 ) ) ;
#5260=CARTESIAN_POINT ( 'NONE',  ( -3.530552100319642062, -292.6047140820548975, -337.1349946108709332 ) ) ;
#5261=CARTESIAN_POINT ( 'NONE',  ( 19.04861993276122334, -280.0368671646253915, -218.1663804704797087 ) ) ;
#5262=CARTESIAN_POINT ( 'NONE',  ( -69.85430415644619018, -289.1237833571632905, -202.7746430608542312 ) ) ;
#5263=CARTESIAN_POINT ( 'NONE',  ( -81.46536161355449224, -277.4522125437222826, -209.6502380899620448 ) ) ;
#5265=CARTESIAN_POINT ( 'NONE',  ( 20.66185906647868009, -286.9773011838267962, -315.3560944145764324 ) ) ;
#5267=CARTESIAN_POINT ( 'NONE',  ( -31.74690424450655257, -286.9815068649705836, -345.2041627897999092 ) ) ;
#5268=CARTESIAN_POINT ( 'NONE',  ( -106.9677340600781719, -274.3903420936792372, -246.2173164837208788 ) ) ;
#5269=CARTESIAN_POINT ( 'NONE',  ( 24.64004677047517688, -283.5747196372540770, -315.0696793122694999 ) ) ;
#5270=CARTESIAN_POINT ( 'NONE',  ( -86.37251689046662761, -295.3960015251328173, -213.0701010210297284 ) ) ;
#5271=CARTESIAN_POINT ( 'NONE',  ( -10.97576954368039281, -282.6987544827048282, -338.4869961247281367 ) ) ;
#5272=CARTESIAN_POINT ( 'NONE',  ( -107.1654792193143209, -296.3033935784346227, -302.8209374198731325 ) ) ;
#5273=CARTESIAN_POINT ( 'NONE',  ( -19.14332126376245924, -275.7161078297808672, -199.0047371827268989 ) ) ;
#5274=ADVANCED_FACE ( 'NONE', ( #55032 ), #61675, .T. ) ;
#5275=CARTESIAN_POINT ( 'NONE',  ( -28.48707960741623779, -282.1645066143585154, -195.8334127119177595 ) ) ;
#5276=CARTESIAN_POINT ( 'NONE',  ( -62.12130349818226449, -272.6425182354039976, -201.3669346750759814 ) ) ;
#5279=CARTESIAN_POINT ( 'NONE',  ( -90.85932714116731290, -287.2685433942630766, -218.2512526014591288 ) ) ;
#5281=CARTESIAN_POINT ( 'NONE',  ( -72.08107566293803359, -280.9809262143061233, -342.4248175857292154 ) ) ;
#5282=CARTESIAN_POINT ( 'NONE',  ( 22.50877645201168775, -275.3967288862177725, -318.5698841057868549 ) ) ;
#5283=CARTESIAN_POINT ( 'NONE',  ( -96.68008155568388418, -288.3042699592049871, -318.1875266655496830 ) ) ;
#5284=CARTESIAN_POINT ( 'NONE',  ( 1.482886347176642916, -284.0435842339068699, -333.0574373803631261 ) ) ;
#5285=CARTESIAN_POINT ( 'NONE',  ( 36.49962194794189685, -277.1681676833748611, -271.5780437319207863 ) ) ;
#5286=CARTESIAN_POINT ( 'NONE',  ( -90.01868687429387705, -285.2038171771376369, -325.7847237581958098 ) ) ;
#5287=CARTESIAN_POINT ( 'NONE',  ( -64.21496463350074180, -282.2056965375770119, -338.6616169552266342 ) ) ;
#5288=CARTESIAN_POINT ( 'NONE',  ( -41.17828725710715787, -282.0040053105010998, -195.4593072585497566 ) ) ;
#5289=CARTESIAN_POINT ( 'NONE',  ( 25.32566527835263415, -275.1259179101189147, -225.5970684731211122 ) ) ;
#5290=CARTESIAN_POINT ( 'NONE',  ( -5.286710171318011575, -276.4751811931974430, -340.3716716398613471 ) ) ;
#5291=CARTESIAN_POINT ( 'NONE',  ( -95.04353818618180583, -297.8192248956215167, -317.4110504620380198 ) ) ;
#5295=CARTESIAN_POINT ( 'NONE',  ( -110.0370414881171683, -294.4190859538852010, -291.7538915127541941 ) ) ;
#5296=CARTESIAN_POINT ( 'NONE',  ( 32.57345518704996579, -275.3409294778575713, -291.6143659916387492 ) ) ;
#5297=CARTESIAN_POINT ( 'NONE',  ( -107.7188072567710719, -274.1460712722865765, -239.9767597071144678 ) ) ;
#5298=CARTESIAN_POINT ( 'NONE',  ( -70.45564045160305966, -287.3696726531240984, -204.1545245047784647 ) ) ;
#5299=CARTESIAN_POINT ( 'NONE',  ( -4.780657072364705940, -296.1512011368319577, -339.3862285684300559 ) ) ;
#5300=CARTESIAN_POINT ( 'NONE',  ( 34.08680801337862931, -295.1096635732735649, -298.0374064336642164 ) ) ;
#5301=CARTESIAN_POINT ( 'NONE',  ( -110.7318267556138380, -292.3632559638281236, -285.0524782475109760 ) ) ;
#5302=CARTESIAN_POINT ( 'NONE',  ( -19.06268687909400938, -278.2876494363108009, -197.7409463991642440 ) ) ;
#5303=CARTESIAN_POINT ( 'NONE',  ( -107.6156734240441040, -280.1501799898020408, -295.0709707241914543 ) ) ;
#5304=CARTESIAN_POINT ( 'NONE',  ( -50.75420014284742365, -293.3046590848770165, -343.5828295067826730 ) ) ;
#5305=CARTESIAN_POINT ( 'NONE',  ( -103.3293793018332138, -285.9203687504344202, -307.6954243731157703 ) ) ;
#5307=CARTESIAN_POINT ( 'NONE',  ( -110.1815076175084585, -283.3579237937252060, -279.0815336135114535 ) ) ;
#5308=CARTESIAN_POINT ( 'NONE',  ( -110.0473503940864930, -271.6917881263019012, -296.1273617737030577 ) ) ;
#5310=CARTESIAN_POINT ( 'NONE',  ( -91.53406346403252769, -284.9202847882768310, -221.3452768021823260 ) ) ;
#5312=CARTESIAN_POINT ( 'NONE',  ( 38.87396411916250116, -282.5189526487523608, -261.3724883060169759 ) ) ;
#5313=CARTESIAN_POINT ( 'NONE',  ( -54.22054209415002646, -274.1626177260037025, -199.3175244602573173 ) ) ;
#5314=CARTESIAN_POINT ( 'NONE',  ( 7.324919880927524218, -285.4406511824274730, -208.0631346806515580 ) ) ;
#5315=CARTESIAN_POINT ( 'NONE',  ( 36.75474168312183565, -282.2408048821324087, -250.2479611428562976 ) ) ;
#5317=CARTESIAN_POINT ( 'NONE',  ( -38.51471153295933902, -278.5867254522245844, -346.6587706291866198 ) ) ;
#5318=CARTESIAN_POINT ( 'NONE',  ( -39.59259826508326796, -280.6760255355429194, -193.4829674633712386 ) ) ;
#5319=CARTESIAN_POINT ( 'NONE',  ( 7.399455738971487229, -273.9094976428776818, -326.5171145203363494 ) ) ;
#5320=CARTESIAN_POINT ( 'NONE',  ( 181.2799904727868352, 253.4939824462867364, -166.7132491217169843 ) ) ;
#5321=ORIENTED_EDGE ( 'NONE', *, *, #12669, .T. ) ;
#5322=CARTESIAN_POINT ( 'NONE',  ( -2.071526431276085933, -276.5204772860475373, -204.3607901335707595 ) ) ;
#5323=CARTESIAN_POINT ( 'NONE',  ( -71.73047451313226475, -195.8125573074262320, -360.1139850430408842 ) ) ;
#5324=CARTESIAN_POINT ( 'NONE',  ( -82.25794907317636273, -277.4564258351906574, -210.6776309431293157 ) ) ;
#5325=CARTESIAN_POINT ( 'NONE',  ( 25.64026602020151557, -294.7435763937052116, -227.7568810026740493 ) ) ;
#5326=CARTESIAN_POINT ( 'NONE',  ( -15.57036931152944348, -294.1115582714140260, -340.1990432870587142 ) ) ;
#5327=CARTESIAN_POINT ( 'NONE',  ( -47.72887221007668046, -291.4312438399701364, -194.0732959488273650 ) ) ;
#5329=CARTESIAN_POINT ( 'NONE',  ( -113.7485848359758052, -295.1365963688830902, -269.5902350348989103 ) ) ;
#5330=CARTESIAN_POINT ( 'NONE',  ( 14.63249618918095329, -286.7051889140808498, -322.7550425499727567 ) ) ;
#5331=CARTESIAN_POINT ( 'NONE',  ( -27.97356497270183340, -294.0326162983287759, -196.6677879158840483 ) ) ;
#5332=CARTESIAN_POINT ( 'NONE',  ( -102.1986019281562506, -285.3981382085561904, -305.0356372421797460 ) ) ;
#5334=CARTESIAN_POINT ( 'NONE',  ( -94.54400060558164398, -292.1899173502172857, -219.1681786911219945 ) ) ;
#5335=CARTESIAN_POINT ( 'NONE',  ( -7.222384578328121307, -283.1384495367122440, -336.9392131542515472 ) ) ;
#5336=CARTESIAN_POINT ( 'NONE',  ( -70.64916894309862982, -294.2765031386915666, -339.3583148291201042 ) ) ;
#5337=CARTESIAN_POINT ( 'NONE',  ( -96.46119502493560560, -292.0165304725848614, -221.2587668399353333 ) ) ;
#5339=CARTESIAN_POINT ( 'NONE',  ( -109.8054730980372824, -290.7160977664470920, -296.3749465954792868 ) ) ;
#5340=CARTESIAN_POINT ( 'NONE',  ( 2.445237189648779452, -286.7686396996656981, -209.1565460669851575 ) ) ;
#5343=CARTESIAN_POINT ( 'NONE',  ( -61.18008840841613249, -297.2186916809318973, -342.3328296288072465 ) ) ;
#5344=CARTESIAN_POINT ( 'NONE',  ( -89.26126760057414344, -296.0247453402004680, -214.0963366250190916 ) ) ;
#5346=CARTESIAN_POINT ( 'NONE',  ( -34.29156781518683772, -279.1501475899522120, -197.1767831543928367 ) ) ;
#5347=CARTESIAN_POINT ( 'NONE',  ( 39.25667566103889783, -274.9625749795221168, -262.5927961482430533 ) ) ;
#5348=CARTESIAN_POINT ( 'NONE',  ( -110.4212285597121053, -295.1610837239347802, -260.4848094460849666 ) ) ;
#5349=CARTESIAN_POINT ( 'NONE',  ( -0.8426005758628622999, -278.4228405349111881, -335.0620155825519646 ) ) ;
#5350=CARTESIAN_POINT ( 'NONE',  ( 36.32890189270359116, -273.8155789671689035, -279.9082986004372060 ) ) ;
#5351=CARTESIAN_POINT ( 'NONE',  ( -39.68643072259058613, -296.2872962933840313, -343.7332287316596080 ) ) ;
#5352=CARTESIAN_POINT ( 'NONE',  ( -110.5216669720627323, -297.6889654293551644, -266.0115748391735337 ) ) ;
#5354=CARTESIAN_POINT ( 'NONE',  ( -65.29090283272493878, -297.0115294369232402, -341.2644173104876586 ) ) ;
#5355=CARTESIAN_POINT ( 'NONE',  ( -48.66797751146319939, -295.9082238656515074, -196.0002937002164742 ) ) ;
#5356=CARTESIAN_POINT ( 'NONE',  ( -14.82287014040335826, -293.0031986035471050, -200.8140478502934343 ) ) ;
#5357=CARTESIAN_POINT ( 'NONE',  ( -27.02833669220459711, -274.9827864666995083, -194.1645582188364472 ) ) ;
#5358=CARTESIAN_POINT ( 'NONE',  ( -98.78156256493859644, -289.6852307859175539, -229.7652793455930009 ) ) ;
#5360=CARTESIAN_POINT ( 'NONE',  ( -93.13186485208019860, -273.7692995974663859, -217.3609085561436132 ) ) ;
#5361=CARTESIAN_POINT ( 'NONE',  ( -109.8249371968531847, -296.7634263136923778, -279.6127325257144207 ) ) ;
#5362=CARTESIAN_POINT ( 'NONE',  ( -68.02635420380981657, -281.6312122117402623, -201.5221955242890601 ) ) ;
#5363=CARTESIAN_POINT ( 'NONE',  ( 36.00108747718874014, -280.5140070920198241, -292.3178449648257811 ) ) ;
#5364=CARTESIAN_POINT ( 'NONE',  ( -59.64338359323848948, -276.6822308723493506, -343.9542406296511672 ) ) ;
#5365=CARTESIAN_POINT ( 'NONE',  ( -31.11855801764535556, -278.5292702933902547, -194.3635146443127155 ) ) ;
#5366=CARTESIAN_POINT ( 'NONE',  ( -8.760165897447723893, -280.6790647664868743, -339.9369770354172715 ) ) ;
#5367=CARTESIAN_POINT ( 'NONE',  ( -3.820204120759785216, -273.0780751921286651, -204.8360230235449819 ) ) ;
#5368=CARTESIAN_POINT ( 'NONE',  ( -66.06938119186142444, -279.4282279167829302, -339.6548854248234193 ) ) ;
#5369=DIRECTION ( 'NONE',  ( 0.000000000000000000, 0.000000000000000000, 1.000000000000000000 ) ) ;
#5371=CARTESIAN_POINT ( 'NONE',  ( -86.78567027478609930, -295.6157171324484239, -212.5919637838878202 ) ) ;
#5372=CARTESIAN_POINT ( 'NONE',  ( -81.93038353165945864, -291.4628157562380579, -207.5849337059135564 ) ) ;
#5373=CARTESIAN_POINT ( 'NONE',  ( 18.53191428103235694, -278.2515910845187364, -320.6612753712871040 ) ) ;
#5374=CARTESIAN_POINT ( 'NONE',  ( 33.00276351448015077, -273.2143846640282163, -244.3484848610641222 ) ) ;
#5376=CARTESIAN_POINT ( 'NONE',  ( -47.04672718844631873, -285.0946683416601672, -345.2952667143387089 ) ) ;
#5379=CARTESIAN_POINT ( 'NONE',  ( 14.13724810170774049, -284.7744174194888842, -215.7481882933411725 ) ) ;
#5382=CARTESIAN_POINT ( 'NONE',  ( 34.45278755785228242, -292.5479999952818844, -285.6752637591023358 ) ) ;
#5383=CARTESIAN_POINT ( 'NONE',  ( 0.8236945865196418914, -284.7061900439438773, -206.6280435039859640 ) ) ;
#5384=CARTESIAN_POINT ( 'NONE',  ( -108.4555765497910471, -262.4588243622614527, -317.8183916042563055 ) ) ;
#5385=CARTESIAN_POINT ( 'NONE',  ( -73.09996504551138230, -293.5259162875414063, -336.3026119318203655 ) ) ;
#5386=CARTESIAN_POINT ( 'NONE',  ( 17.86340071275525077, -285.3044799336849451, -217.6056316480299131 ) ) ;
#5387=CARTESIAN_POINT ( 'NONE',  ( -30.20508680632367771, -281.7439312431374674, -196.8560815410151008 ) ) ;
#5388=CARTESIAN_POINT ( 'NONE',  ( -15.54122839912241361, -287.5331199298364027, -196.8706820252133127 ) ) ;
#5389=CARTESIAN_POINT ( 'NONE',  ( 17.08460742235845942, -280.5294678211956239, -323.4622253411221777 ) ) ;
#5390=CARTESIAN_POINT ( 'NONE',  ( 21.17348472762059330, -288.1647967497415266, -314.0280409378009381 ) ) ;
#5391=CARTESIAN_POINT ( 'NONE',  ( -109.4683650643524686, -280.1692941665662033, -255.6991640077160355 ) ) ;
#5392=CARTESIAN_POINT ( 'NONE',  ( 9.371802247482049708, -281.5159353667501705, -213.9883327953642436 ) ) ;
#5393=CARTESIAN_POINT ( 'NONE',  ( -86.69220583825989479, -287.3504050384118500, -213.3452500646500596 ) ) ;
#5395=CARTESIAN_POINT ( 'NONE',  ( -70.72712248506790900, -297.4572214226643609, -200.9751426086801303 ) ) ;
#5396=CARTESIAN_POINT ( 'NONE',  ( -111.3339271812367741, -292.6640637999180967, -260.1280646640802843 ) ) ;
#5398=CARTESIAN_POINT ( 'NONE',  ( -19.05039376806008633, -291.3376638359844719, -350.3538533559490702 ) ) ;
#5400=CARTESIAN_POINT ( 'NONE',  ( -77.83203036665101138, -271.5094251223428046, -207.0321231828860391 ) ) ;
#5402=CARTESIAN_POINT ( 'NONE',  ( -100.9715923828847650, -294.3939081936653679, -312.3812434406018497 ) ) ;
#5403=CARTESIAN_POINT ( 'NONE',  ( -104.4700245547546444, -272.2906577436394855, -241.2901558669481119 ) ) ;
#5404=CARTESIAN_POINT ( 'NONE',  ( -20.95653174262839968, -290.3581722686908506, -342.2098062619330676 ) ) ;
#5405=CARTESIAN_POINT ( 'NONE',  ( 36.14870698110495084, -283.4320157171180767, -279.5622748089360243 ) ) ;
#5406=CARTESIAN_POINT ( 'NONE',  ( -89.07908564030039145, -291.1882201889321209, -326.5914410473200178 ) ) ;
#5407=CARTESIAN_POINT ( 'NONE',  ( -38.89327520837697705, -290.3864045160495948, -346.8522343896697748 ) ) ;
#5408=CARTESIAN_POINT ( 'NONE',  ( -93.02270218098389876, -287.2533497275067020, -220.0391129598299926 ) ) ;
#5409=CARTESIAN_POINT ( 'NONE',  ( -1.137313172042173637, -280.6857841603659836, -202.4034666866361079 ) ) ;
#5410=CARTESIAN_POINT ( 'NONE',  ( -76.35998312317518355, -293.6489906156095344, -335.1281645716942990 ) ) ;
#5411=CARTESIAN_POINT ( 'NONE',  ( -18.92045261105681320, -282.6547958653488308, -345.1800883678939726 ) ) ;
#5412=CARTESIAN_POINT ( 'NONE',  ( 36.87735890785094028, -277.3924924266790981, -268.8129728632264914 ) ) ;
#5413=CARTESIAN_POINT ( 'NONE',  ( -69.91165696735023971, -300.1233781216987495, -202.8022627189028810 ) ) ;
#5414=CARTESIAN_POINT ( 'NONE',  ( 22.70334180902946741, -274.4223787587929451, -316.9500878260288346 ) ) ;
#5416=CARTESIAN_POINT ( 'NONE',  ( 24.17887476714351180, -281.6056657105210661, -309.8648626097793226 ) ) ;
#5417=CARTESIAN_POINT ( 'NONE',  ( -72.64397219414360052, -278.7140798856932520, -338.3592596393396548 ) ) ;
#5418=CARTESIAN_POINT ( 'NONE',  ( -64.45284291391246256, -284.7655590847701319, -198.5291267034803013 ) ) ;
#5419=CARTESIAN_POINT ( 'NONE',  ( -25.26553288692907984, -293.9682054081092701, -197.2874221465583844 ) ) ;
#5420=CARTESIAN_POINT ( 'NONE',  ( -85.32047880293654885, -275.0018201955659265, -211.1624929118229090 ) ) ;
#5421=CARTESIAN_POINT ( 'NONE',  ( -69.93698448296969161, -274.9470042999743669, -201.1308603885958348 ) ) ;
#5423=CARTESIAN_POINT ( 'NONE',  ( 35.69880132918699189, -275.4016435397434179, -271.5870845242342853 ) ) ;
#5424=CARTESIAN_POINT ( 'NONE',  ( -109.7368646091377542, -298.3076993834943096, -289.3581808543477791 ) ) ;
#5425=CARTESIAN_POINT ( 'NONE',  ( -112.1526875629296711, -282.5090842962747502, -273.6950319864021708 ) ) ;
#5426=CARTESIAN_POINT ( 'NONE',  ( -40.62726875816204597, -291.6786425977870181, -193.4392316050483771 ) ) ;
#5427=CARTESIAN_POINT ( 'NONE',  ( 34.44875389110028863, -273.3057524237379425, -249.7317006916813966 ) ) ;
#5428=CARTESIAN_POINT ( 'NONE',  ( 2.776458437701260440, -290.1239836843585636, -335.2070805235773037 ) ) ;
#5429=CARTESIAN_POINT ( 'NONE',  ( -91.89402461993891791, -290.1706027301854078, -221.3702116796339965 ) ) ;
#5431=CARTESIAN_POINT ( 'NONE',  ( -1.067456681578598188, -291.0987168241476297, -203.1094595924608086 ) ) ;
#5432=CARTESIAN_POINT ( 'NONE',  ( -109.2968560456548346, -290.3866207179117964, -257.6409832619119697 ) ) ;
#5434=CARTESIAN_POINT ( 'NONE',  ( 35.65775334262585972, -288.9286167610696339, -293.8679744847405573 ) ) ;
#5435=CARTESIAN_POINT ( 'NONE',  ( -69.75349940843321406, -279.9464838182449853, -204.9136165103991516 ) ) ;
#5436=CARTESIAN_POINT ( 'NONE',  ( -70.68595502335614356, -294.4018871641715123, -339.4382465362657513 ) ) ;
#5437=CARTESIAN_POINT ( 'NONE',  ( -40.82017651476156317, -286.6610198230948185, -193.4896414072865127 ) ) ;
#5438=CARTESIAN_POINT ( 'NONE',  ( -104.0242643699765068, -285.3867409809321316, -231.7949971845740720 ) ) ;
#5439=CARTESIAN_POINT ( 'NONE',  ( -18.72615083281375803, -283.1391653318508475, -341.0219569492464871 ) ) ;
#5440=CARTESIAN_POINT ( 'NONE',  ( -63.77599425757506424, -182.7598565315317671, -362.4607550793396626 ) ) ;
#5441=CARTESIAN_POINT ( 'NONE',  ( -108.4164688561979517, -260.9275896293593178, -316.9037050568759923 ) ) ;
#5442=CARTESIAN_POINT ( 'NONE',  ( -83.63476906808553224, -218.2911303493422395, -349.0134962854843934 ) ) ;
#5443=CARTESIAN_POINT ( 'NONE',  ( 34.28152331167102318, -274.5520784815808497, -255.3762593438608235 ) ) ;
#5444=CARTESIAN_POINT ( 'NONE',  ( 32.80819680017828688, -274.7537000723331744, -291.6935245946856980 ) ) ;
#5445=CARTESIAN_POINT ( 'NONE',  ( -111.9105587548108787, -295.8219239643988772, -289.3619402754126213 ) ) ;
#5446=CARTESIAN_POINT ( 'NONE',  ( 38.24303543357504509, -274.0868555633581991, -258.4340045478792831 ) ) ;
#5447=CARTESIAN_POINT ( 'NONE',  ( -79.44974825397535767, -275.2353816569271316, -209.4310739421757717 ) ) ;
#5449=CARTESIAN_POINT ( 'NONE',  ( -106.3072007313882068, -297.9276384897456182, -236.6479167282529943 ) ) ;
#5451=CARTESIAN_POINT ( 'NONE',  ( 24.29362433334187088, -288.5864708224853530, -309.5921671675813514 ) ) ;
#5452=CARTESIAN_POINT ( 'NONE',  ( -113.9606668629597124, -297.4360301119655219, -263.8942465129169364 ) ) ;
#5453=CARTESIAN_POINT ( 'NONE',  ( -84.14279676444506606, -296.1682557354691880, -331.4953327629798991 ) ) ;
#5454=CARTESIAN_POINT ( 'NONE',  ( 19.34444822530857877, -293.0678533609273586, -224.3448204923146818 ) ) ;
#5456=CARTESIAN_POINT ( 'NONE',  ( 23.30912041543534485, -276.8616581992542933, -225.2968065162450557 ) ) ;
#5458=CARTESIAN_POINT ( 'NONE',  ( 3.794371498737300730, -280.0973272094233266, -205.2801054081666621 ) ) ;
#5459=CARTESIAN_POINT ( 'NONE',  ( -18.94630583136317625, -277.7507182464654534, -341.2484787464994156 ) ) ;
#5460=CARTESIAN_POINT ( 'NONE',  ( -10.72386229093856613, -276.1545851966166651, -199.1330697768378855 ) ) ;
#5461=CARTESIAN_POINT ( 'NONE',  ( -67.08314674709232861, -275.4602061078032875, -339.5987750625994295 ) ) ;
#5462=CARTESIAN_POINT ( 'NONE',  ( -33.81423868219317086, -298.7488730663218917, -197.2587812560099394 ) ) ;
#5463=CARTESIAN_POINT ( 'NONE',  ( -72.42131744404025540, -294.1007116034472233, -335.0654981178685148 ) ) ;
#5464=CARTESIAN_POINT ( 'NONE',  ( -36.75932130260467545, -280.5516329904406234, -193.4118253768584452 ) ) ;
#5465=CARTESIAN_POINT ( 'NONE',  ( 31.26249086718059544, -276.0530131352813896, -295.4572700622679804 ) ) ;
#5466=CARTESIAN_POINT ( 'NONE',  ( -33.73372242345659799, -284.7814962261444975, -193.9393882819498174 ) ) ;
#5467=CARTESIAN_POINT ( 'NONE',  ( -106.2502911651721433, -274.9410280725825828, -240.6221293452589123 ) ) ;
#5469=CARTESIAN_POINT ( 'NONE',  ( 27.80657692643085355, -286.2966790643522472, -236.9581922654245432 ) ) ;
#5470=CARTESIAN_POINT ( 'NONE',  ( -3.869513343373986114, -278.7397397698162536, -204.3350128375695647 ) ) ;
#5471=CARTESIAN_POINT ( 'NONE',  ( -72.39452319863323737, -278.1533155698182895, -205.6566010391548218 ) ) ;
#5472=CARTESIAN_POINT ( 'NONE',  ( -85.81768114545829462, -281.8094876236396544, -326.8535374694505435 ) ) ;
#5473=CARTESIAN_POINT ( 'NONE',  ( 34.36810695736087240, -289.2670677736219318, -248.2169718605323681 ) ) ;
#5474=CARTESIAN_POINT ( 'NONE',  ( -87.35494975445554644, -278.9736733063753604, -324.0808105156456236 ) ) ;
#5476=CARTESIAN_POINT ( 'NONE',  ( -73.73139976847886601, -293.5691591426621585, -204.7807061948793717 ) ) ;
#5477=CARTESIAN_POINT ( 'NONE',  ( -34.35367924942621443, -275.2549317083983169, -346.2890163253703690 ) ) ;
#5478=CARTESIAN_POINT ( 'NONE',  ( 33.34287402041501025, -276.4494048833050783, -289.0047132877681975 ) ) ;
#5479=CARTESIAN_POINT ( 'NONE',  ( 37.78819233731191218, -283.5824370664340108, -272.7122202209787361 ) ) ;
#5481=CARTESIAN_POINT ( 'NONE',  ( -45.83908004566023209, -291.0790993861033371, -345.4939320029951091 ) ) ;
#5482=CARTESIAN_POINT ( 'NONE',  ( -88.63569068191966949, -295.3328101065662281, -215.5740016657954072 ) ) ;
#5483=CARTESIAN_POINT ( 'NONE',  ( -43.64280885152134459, -285.1717589438429172, -193.7282419513626053 ) ) ;
#5484=CARTESIAN_POINT ( 'NONE',  ( 7.645911783477549406, -273.3659203075015398, -212.2460747401012497 ) ) ;
#5485=CARTESIAN_POINT ( 'NONE',  ( -5.490531708281201517, -290.6152415047042155, -203.2921336742650169 ) ) ;
#5488=CARTESIAN_POINT ( 'NONE',  ( -71.84132664023964310, -290.0844397742574188, -202.2843013960701626 ) ) ;
#5489=CARTESIAN_POINT ( 'NONE',  ( -98.18041534171183571, -285.5759949885751325, -312.2244383742435048 ) ) ;
#5490=CARTESIAN_POINT ( 'NONE',  ( -29.54433916542513927, -284.3894837741799506, -194.7755692647185128 ) ) ;
#5491=CARTESIAN_POINT ( 'NONE',  ( -71.46745531407400165, -287.0173803292636308, -205.1628990541616702 ) ) ;
#5492=CARTESIAN_POINT ( 'NONE',  ( -39.98997923783336716, -286.8208628645006684, -197.2475874624307437 ) ) ;
#5493=CARTESIAN_POINT ( 'NONE',  ( -106.8596758165687959, -292.9099816220318644, -241.2809210038930701 ) ) ;
#5494=CARTESIAN_POINT ( 'NONE',  ( 15.92245980209379397, -274.3848484328967174, -324.0274687671739002 ) ) ;
#5495=CARTESIAN_POINT ( 'NONE',  ( -2.730813788030802325, -276.9404789673832852, -339.1350159257519863 ) ) ;
#5496=CARTESIAN_POINT ( 'NONE',  ( 29.63407067054737709, -291.1708336987174448, -235.2689848466014837 ) ) ;
#5497=CARTESIAN_POINT ( 'NONE',  ( -97.69689608917815349, -279.1919871590289404, -222.5463679518675235 ) ) ;
#5498=CARTESIAN_POINT ( 'NONE',  ( -34.20745176364884088, -296.9924347345354363, -344.9400915079979768 ) ) ;
#5501=CARTESIAN_POINT ( 'NONE',  ( -106.6443321494666492, -282.9118259216588740, -294.9747467497087428 ) ) ;
#5503=CARTESIAN_POINT ( 'NONE',  ( -3.275213607004501259, -278.5018131557751531, -203.5300427465863891 ) ) ;
#5506=CARTESIAN_POINT ( 'NONE',  ( -35.52075116320298065, -272.5544647369757740, -194.0631673642092210 ) ) ;
#5507=CARTESIAN_POINT ( 'NONE',  ( -45.92829389768586879, -276.5123475911731248, -343.0077035009559836 ) ) ;
#5509=CARTESIAN_POINT ( 'NONE',  ( 25.02425220122042404, -295.6105815909129433, -309.7150785287620351 ) ) ;
#5510=CARTESIAN_POINT ( 'NONE',  ( 36.30673496341573525, -280.2026744850689397, -248.9270851843121193 ) ) ;
#5511=CARTESIAN_POINT ( 'NONE',  ( -4.219553271621838242, -295.5456506989467584, -335.6923256632015864 ) ) ;
#5512=CARTESIAN_POINT ( 'NONE',  ( -30.61750492614311270, -296.2839782419682706, -346.5719011530021589 ) ) ;
#5513=CARTESIAN_POINT ( 'NONE',  ( -108.5545752497937002, -272.4318502960808246, -254.2113841215606840 ) ) ;
#5514=CARTESIAN_POINT ( 'NONE',  ( -109.3217578038006508, -292.8241350142209853, -249.2471933768260897 ) ) ;
#5515=CARTESIAN_POINT ( 'NONE',  ( -3.491271147477023717, -286.6533402012302076, -201.1862804223633532 ) ) ;
#5516=CARTESIAN_POINT ( 'NONE',  ( 28.87963451420861816, -273.2055822605782964, -233.4423032827533859 ) ) ;
#5517=CARTESIAN_POINT ( 'NONE',  ( 32.86400680427562548, -287.7894348986568502, -301.9864040462904313 ) ) ;
#5518=CARTESIAN_POINT ( 'NONE',  ( -41.15997995227332495, -281.9837402886147970, -195.8140352522186447 ) ) ;
#5519=CARTESIAN_POINT ( 'NONE',  ( -102.4420922380332115, -284.0654762150477382, -236.8149200678552120 ) ) ;
#5520=CARTESIAN_POINT ( 'NONE',  ( -111.6801955450985417, -288.6844786863240415, -260.0426056375736152 ) ) ;
#5521=CARTESIAN_POINT ( 'NONE',  ( 197.2116108777964030, 281.1590520725322335, -110.1526527170710921 ) ) ;
#5522=CARTESIAN_POINT ( 'NONE',  ( -49.42553807858669046, -285.4017234780982903, -198.2542556404781635 ) ) ;
#5524=CARTESIAN_POINT ( 'NONE',  ( 38.43750813057442883, -282.6482423518629048, -282.7042943749214032 ) ) ;
#5525=CARTESIAN_POINT ( 'NONE',  ( -88.48377956138980949, -290.4142143431329828, -213.1133414004349902 ) ) ;
#5526=CARTESIAN_POINT ( 'NONE',  ( -113.4133967445942659, -280.2081394517334729, -265.9410062684237346 ) ) ;
#5527=CARTESIAN_POINT ( 'NONE',  ( -113.8847771688643604, -279.8874608218376352, -268.7613794830327834 ) ) ;
#5528=CARTESIAN_POINT ( 'NONE',  ( 29.31359241368011581, -281.7877946511563323, -300.2521860480696887 ) ) ;
#5529=CARTESIAN_POINT ( 'NONE',  ( -21.53673754881911506, -276.2549749414772009, -197.0453365742241374 ) ) ;
#5530=CARTESIAN_POINT ( 'NONE',  ( -11.05720881478716677, -294.7189562055155534, -342.7925829689958164 ) ) ;
#5531=CARTESIAN_POINT ( 'NONE',  ( -69.70849848579398156, -289.6440886384245346, -203.0845556857270822 ) ) ;
#5532=CARTESIAN_POINT ( 'NONE',  ( -83.42806130488330041, -272.1987623064530908, -213.2368865471187291 ) ) ;
#5534=CARTESIAN_POINT ( 'NONE',  ( -15.69077336091294050, -284.6899837677090090, -341.5829655140714749 ) ) ;
#5535=CARTESIAN_POINT ( 'NONE',  ( -88.51969505725719500, -295.4605489573743853, -322.5176916312478284 ) ) ;
#5536=CARTESIAN_POINT ( 'NONE',  ( 1.531509762563444621, -293.6382648281865499, -204.1916902035282249 ) ) ;
#5537=CARTESIAN_POINT ( 'NONE',  ( 1.162039982135356198, -283.1750155104984970, -332.5600293800106897 ) ) ;
#5538=CARTESIAN_POINT ( 'NONE',  ( 11.64478784276426460, -273.7713977941410235, -211.1892083145288268 ) ) ;
#5539=CARTESIAN_POINT ( 'NONE',  ( -101.6033493867251707, -291.7605700994229778, -228.0310465856279620 ) ) ;
#5540=CARTESIAN_POINT ( 'NONE',  ( -73.01021708519841980, -283.7246118193895654, -203.4594523454158264 ) ) ;
#5541=CARTESIAN_POINT ( 'NONE',  ( -89.47404530119399624, -290.0964049248355536, -326.9999993115879988 ) ) ;
#5543=CARTESIAN_POINT ( 'NONE',  ( 32.68904205201485524, -287.6113037408824198, -249.6341109729900438 ) ) ;
#5546=CARTESIAN_POINT ( 'NONE',  ( 184.5454089206492370, 260.5126890106757855, -150.9870170413777259 ) ) ;
#5547=CARTESIAN_POINT ( 'NONE',  ( -70.15427116186016576, -284.9966942577644318, -339.2669782279853052 ) ) ;
#5548=CARTESIAN_POINT ( 'NONE',  ( -85.33152481854864391, -287.1952119285919025, -330.4860931364850671 ) ) ;
#5550=CARTESIAN_POINT ( 'NONE',  ( -4.701833389319127754, -281.5320240312600504, -336.0030647383991322 ) ) ;
#5551=CARTESIAN_POINT ( 'NONE',  ( -25.77733502521724063, -276.5753990247985712, -346.4663724083969782 ) ) ;
#5552=CARTESIAN_POINT ( 'NONE',  ( -103.4652757070050484, -280.0867013984362188, -305.3996849660924227 ) ) ;
#5553=CARTESIAN_POINT ( 'NONE',  ( 195.3697669529573488, 276.2562599343855823, -124.8324474917287006 ) ) ;
#5554=CARTESIAN_POINT ( 'NONE',  ( 33.01622799889876347, -280.5106917123473522, -300.3016712754254058 ) ) ;
#5555=CARTESIAN_POINT ( 'NONE',  ( -95.38547903890790280, -283.2216319223433629, -223.4072294020228071 ) ) ;
#5556=CARTESIAN_POINT ( 'NONE',  ( -105.0445240052205520, -297.8607417579097500, -304.9777072601681880 ) ) ;
#5557=CARTESIAN_POINT ( 'NONE',  ( 10.96680164365356092, -293.2341867575362926, -215.4823279046650555 ) ) ;
#5559=CARTESIAN_POINT ( 'NONE',  ( -106.5022732242845365, -288.9081005424685600, -295.2219024927940723 ) ) ;
#5560=CARTESIAN_POINT ( 'NONE',  ( -54.10094124125617299, -277.9131764608919752, -345.4652725364228445 ) ) ;
#5561=CARTESIAN_POINT ( 'NONE',  ( 51.66713944345190157, -299.3636508086932508, -197.3585598630277786 ) ) ;
#5563=CARTESIAN_POINT ( 'NONE',  ( -103.9541965870423610, -271.9692864156799601, -232.2510524344049827 ) ) ;
#5567=CARTESIAN_POINT ( 'NONE',  ( 19.60080703926609758, -283.2825294796509183, -316.5520791792329760 ) ) ;
#5568=CARTESIAN_POINT ( 'NONE',  ( -17.28136713122432155, -282.0677492029905693, -197.0702109645048665 ) ) ;
#5569=CARTESIAN_POINT ( 'NONE',  ( -107.2139281121345391, -283.3210610690902627, -292.2992173708490213 ) ) ;
#5570=CARTESIAN_POINT ( 'NONE',  ( -5.042114974350710987, -282.3424049903294986, -203.5209931847413145 ) ) ;
#5571=CARTESIAN_POINT ( 'NONE',  ( 34.56557363288298035, -274.2435064169627026, -286.5445526688300788 ) ) ;
#5574=CARTESIAN_POINT ( 'NONE',  ( -93.20954401653233390, -278.6324439859234303, -323.1910615350674334 ) ) ;
#5578=CARTESIAN_POINT ( 'NONE',  ( -51.95856947680374560, -287.7275685084561587, -195.9661374918085812 ) ) ;
#5579=CARTESIAN_POINT ( 'NONE',  ( 32.78679680666646590, -292.4719532717985544, -249.3395017370283142 ) ) ;
#5580=CARTESIAN_POINT ( 'NONE',  ( 28.81182572348724591, -287.4122070779985165, -309.5660131331752609 ) ) ;
#5581=CARTESIAN_POINT ( 'NONE',  ( -57.65122327509429567, -284.0263095083828375, -199.1354727095479404 ) ) ;
#5582=CARTESIAN_POINT ( 'NONE',  ( -110.1930058801434313, -283.2629078724136775, -259.9658225330260279 ) ) ;
#5583=CARTESIAN_POINT ( 'NONE',  ( -95.76408712385619992, -288.1603795956080489, -315.8216589771979557 ) ) ;
#5584=CARTESIAN_POINT ( 'NONE',  ( -109.0561512620158595, -285.9630169080711539, -254.6765096224464173 ) ) ;
#5585=CARTESIAN_POINT ( 'NONE',  ( 31.18187667383045891, -273.9515086906824308, -300.8491495366205868 ) ) ;
#5586=CARTESIAN_POINT ( 'NONE',  ( -35.15060753806464788, -284.4790774039164489, -194.1796169645465966 ) ) ;
#5587=CARTESIAN_POINT ( 'NONE',  ( -81.80590019574881921, -299.4471366300478508, -209.8984327494680997 ) ) ;
#5588=CARTESIAN_POINT ( 'NONE',  ( -82.16179362472456660, -283.4427157186805175, -209.9539736317233292 ) ) ;
#5589=CARTESIAN_POINT ( 'NONE',  ( 25.33145975030688390, -281.9723805651395310, -232.3750943571965593 ) ) ;
#5590=CARTESIAN_POINT ( 'NONE',  ( 36.96916418498377510, -289.4063156126323975, -258.9652657521698416 ) ) ;
#5593=CARTESIAN_POINT ( 'NONE',  ( -55.69637267576413109, -297.2067866202677351, -343.6579132117065569 ) ) ;
#5594=CARTESIAN_POINT ( 'NONE',  ( -52.19930863203599358, -277.8619052777128218, -196.7943546940425961 ) ) ;
#5595=CARTESIAN_POINT ( 'NONE',  ( -113.9523537845118426, -289.6670009002696702, -276.9295910252459407 ) ) ;
#5596=CARTESIAN_POINT ( 'NONE',  ( -34.28826986981983538, -293.4129927498764800, -344.0979268381724978 ) ) ;
#5597=CARTESIAN_POINT ( 'NONE',  ( -62.46187359309388398, -278.4033222996719132, -201.2406237979824368 ) ) ;
#5598=CARTESIAN_POINT ( 'NONE',  ( -107.6587733648807017, -270.9506206393151615, -245.9311485109034265 ) ) ;
#5599=CARTESIAN_POINT ( 'NONE',  ( 23.74187897336652497, -294.3035887487042146, -229.4949970229460234 ) ) ;
#5600=CARTESIAN_POINT ( 'NONE',  ( 35.77081079830085031, -295.8376638359844719, -253.6410175316879361 ) ) ;
#5601=CARTESIAN_POINT ( 'NONE',  ( -80.21928799503250218, -295.9632749307266408, -207.1769181385298566 ) ) ;
#5602=CARTESIAN_POINT ( 'NONE',  ( -76.27365832938465928, -291.1822484104104092, -333.0567561500868692 ) ) ;
#5603=CARTESIAN_POINT ( 'NONE',  ( 28.60743337927727126, -291.2950960221364767, -232.6161076970519730 ) ) ;
#5604=CARTESIAN_POINT ( 'NONE',  ( -91.20273039443296170, -292.6927889947307904, -220.1990439280312728 ) ) ;
#5606=CARTESIAN_POINT ( 'NONE',  ( -86.04412536186593741, -292.1595509056815558, -215.6973577332717582 ) ) ;
#5608=CARTESIAN_POINT ( 'NONE',  ( -112.7836469434348601, -291.9242462224384553, -257.0749831088918427 ) ) ;
#5609=CARTESIAN_POINT ( 'NONE',  ( 26.47219683460998851, -279.0349508923584381, -230.1859362376403340 ) ) ;
#5610=CARTESIAN_POINT ( 'NONE',  ( 20.99380109711410114, -292.9358769336175214, -226.4752512735018684 ) ) ;
#5611=CARTESIAN_POINT ( 'NONE',  ( 38.79472841750325074, -281.4040070335026940, -258.5155531832975839 ) ) ;
#5612=CARTESIAN_POINT ( 'NONE',  ( -93.41904383985618665, -283.4987203639658446, -323.1163500267418272 ) ) ;
#5613=CARTESIAN_POINT ( 'NONE',  ( 15.35681882691578970, -286.3052212947831094, -323.4920367141627935 ) ) ;
#5614=CARTESIAN_POINT ( 'NONE',  ( 36.75417371208818196, -279.6327569679189082, -265.8150253872286726 ) ) ;
#5616=CARTESIAN_POINT ( 'NONE',  ( -112.3406650238408844, -282.5570572181266584, -269.9662633438911143 ) ) ;
#5617=CARTESIAN_POINT ( 'NONE',  ( 5.808273747023926070, -279.1054385773423974, -207.4263302586238069 ) ) ;
#5618=CARTESIAN_POINT ( 'NONE',  ( -49.28297903664213919, -284.8238338506865830, -194.5520818110061612 ) ) ;
#5620=CARTESIAN_POINT ( 'NONE',  ( -17.23398796873227212, -293.9160412805918554, -199.3000649083326152 ) ) ;
#5621=CARTESIAN_POINT ( 'NONE',  ( -0.3467466184871222379, -275.9593306577713179, -203.4883343111314957 ) ) ;
#5622=CARTESIAN_POINT ( 'NONE',  ( -93.62504108874649944, -277.5593605828123600, -316.9024582956938048 ) ) ;
#5623=CARTESIAN_POINT ( 'NONE',  ( -79.59619065119146342, -291.6652474566738533, -205.9269059334205281 ) ) ;
#5624=CARTESIAN_POINT ( 'NONE',  ( -66.05217311612736353, -281.5047655090019134, -340.2679799701940624 ) ) ;
#5625=CARTESIAN_POINT ( 'NONE',  ( -88.08500906111720496, -290.3798755850584143, -217.4845594673777214 ) ) ;
#5626=CARTESIAN_POINT ( 'NONE',  ( -105.9333337881992776, -294.9508387465737655, -239.8982049057893562 ) ) ;
#5629=CARTESIAN_POINT ( 'NONE',  ( 18.52769258985101075, -292.3914859456656359, -223.2803427217227465 ) ) ;
#5631=CARTESIAN_POINT ( 'NONE',  ( -37.30987171927208834, -277.5523547857346784, -200.3611179825600459 ) ) ;
#5632=CARTESIAN_POINT ( 'NONE',  ( -108.1626175631348872, -295.2314964713905283, -300.1166098182427504 ) ) ;
#5633=CARTESIAN_POINT ( 'NONE',  ( -11.90142943120043562, -278.5192682303486436, -198.9400814747437778 ) ) ;
#5634=CARTESIAN_POINT ( 'NONE',  ( -95.45303081468092898, -286.5437661329399930, -220.5184870140299722 ) ) ;
#5635=CARTESIAN_POINT ( 'NONE',  ( -30.52916995337177397, -285.9738726731947054, -197.6288951263543936 ) ) ;
#5636=CARTESIAN_POINT ( 'NONE',  ( 3.534619097436099366, -278.0113891344436183, -331.6786055197911196 ) ) ;
#5637=CARTESIAN_POINT ( 'NONE',  ( -67.99316172634625843, -293.4766394464046471, -338.4363924853286676 ) ) ;
#5638=CARTESIAN_POINT ( 'NONE',  ( -109.1636528616686519, -298.5455823196704159, -252.4323348575089199 ) ) ;
#5639=CARTESIAN_POINT ( 'NONE',  ( -83.26710060335335584, -276.4921310575663256, -327.6802575631335799 ) ) ;
#5642=CARTESIAN_POINT ( 'NONE',  ( -88.59451888659819474, -295.4144670288345083, -327.8685909876565461 ) ) ;
#5643=CARTESIAN_POINT ( 'NONE',  ( -91.62643743080401748, -291.7527655932216248, -321.3724185486800593 ) ) ;
#5645=CARTESIAN_POINT ( 'NONE',  ( 3.678657312822051662, -289.1357101857873886, -330.9302009553198900 ) ) ;
#5647=CARTESIAN_POINT ( 'NONE',  ( -28.24096526810764018, -279.2235681044772377, -194.0843210317271144 ) ) ;
#5648=CARTESIAN_POINT ( 'NONE',  ( -93.60921940953377884, -296.4879261976922180, -322.7950019955405310 ) ) ;
#5649=CARTESIAN_POINT ( 'NONE',  ( -107.6609930154991588, -288.3279726715115885, -298.5657723172761848 ) ) ;
#5650=CARTESIAN_POINT ( 'NONE',  ( 99.13515218641353499, -300.0504093806150081, -193.3746630480670206 ) ) ;
#5651=CARTESIAN_POINT ( 'NONE',  ( 25.81307700534236815, -294.3881600115214496, -307.0157440471986661 ) ) ;
#5652=DIRECTION ( 'NONE',  ( -1.000000000000000000, -0.000000000000000000, -0.000000000000000000 ) ) ;
#5654=CARTESIAN_POINT ( 'NONE',  ( 28.31710113668617623, -289.5833924468494729, -309.2407986387399887 ) ) ;
#5655=CARTESIAN_POINT ( 'NONE',  ( 25.18497378105907814, -277.4090924074130839, -220.4570493818173702 ) ) ;
#5656=CARTESIAN_POINT ( 'NONE',  ( 39.17580220988369888, -281.0028635941001767, -278.5159741764853720 ) ) ;
#5657=CARTESIAN_POINT ( 'NONE',  ( -110.7737083985673223, -286.3668230328852360, -284.7752981819294291 ) ) ;
#5658=CARTESIAN_POINT ( 'NONE',  ( 4.869411245364308805, -285.1846773870627203, -206.6048516756858646 ) ) ;
#5659=CARTESIAN_POINT ( 'NONE',  ( -111.4031604879961890, -288.7289859190711354, -262.8634993035025786 ) ) ;
#5660=CARTESIAN_POINT ( 'NONE',  ( 20.79825005036669339, -278.0769382762753708, -318.9414810605923662 ) ) ;
#5661=CARTESIAN_POINT ( 'NONE',  ( -93.60603105028444304, -277.8925878321043683, -316.8922617546468246 ) ) ;
#5662=CARTESIAN_POINT ( 'NONE',  ( 27.87607787754784638, -280.4516509231459622, -237.2256170099288397 ) ) ;
#5663=CARTESIAN_POINT ( 'NONE',  ( 18.68681045751782221, -277.3488972570648343, -322.7280780940164391 ) ) ;
#5664=CARTESIAN_POINT ( 'NONE',  ( -50.85443512913958131, -278.6781054830190669, -194.9594289408277064 ) ) ;
#5665=CARTESIAN_POINT ( 'NONE',  ( 197.4499846583558735, 287.9957563964159704, -96.69947844503649037 ) ) ;
#5666=CARTESIAN_POINT ( 'NONE',  ( -36.95299686282403684, -274.9981862233350398, -193.5843832884686435 ) ) ;
#5668=CARTESIAN_POINT ( 'NONE',  ( -48.89892632017314611, -299.3331050946438268, -194.7761668995491391 ) ) ;
#5669=CARTESIAN_POINT ( 'NONE',  ( 35.78497577281001440, -284.2662352645559167, -287.0191576251351080 ) ) ;
#5671=CARTESIAN_POINT ( 'NONE',  ( 82.66879183539302289, -297.9920280515540867, -193.4024536127582223 ) ) ;
#5672=CARTESIAN_POINT ( 'NONE',  ( 33.32358271772303482, -288.3751082412466076, -250.8510212492540745 ) ) ;
#5673=CARTESIAN_POINT ( 'NONE',  ( 23.87344923371064809, -288.7062910445437751, -225.3424606930140897 ) ) ;
#5674=CARTESIAN_POINT ( 'NONE',  ( 35.73150017091970909, -286.9456784382553565, -273.7728471660273044 ) ) ;
#5675=CARTESIAN_POINT ( 'NONE',  ( -114.2935439285235475, -284.0287668933531791, -272.8409890777389251 ) ) ;
#5676=CARTESIAN_POINT ( 'NONE',  ( -67.61603537093199634, -278.0480659035180224, -203.0427954839507265 ) ) ;
#5677=CARTESIAN_POINT ( 'NONE',  ( 9.796881287871864075, -288.5696808852056279, -213.0128868019011747 ) ) ;
#5678=CARTESIAN_POINT ( 'NONE',  ( 20.22968872378977423, -279.3882652074225916, -224.3584774011443699 ) ) ;
#5679=CARTESIAN_POINT ( 'NONE',  ( -110.7721878770511807, -279.8275744634916009, -273.3954129017844252 ) ) ;
#5680=CARTESIAN_POINT ( 'NONE',  ( -9.959485904892984465, -277.1770588259588521, -338.1109694485344335 ) ) ;
#5682=CARTESIAN_POINT ( 'NONE',  ( -80.33053985741152303, -288.4149961440023162, -333.8284271651554036 ) ) ;
#5683=CARTESIAN_POINT ( 'NONE',  ( -13.46239326642392697, -283.5526043915160699, -343.3949288099326509 ) ) ;
#5684=CARTESIAN_POINT ( 'NONE',  ( -113.5375302539641496, -284.9063148473331921, -281.4012726969455684 ) ) ;
#5685=CARTESIAN_POINT ( 'NONE',  ( 33.32404600059935973, -281.9611809040770254, -288.7235424419137644 ) ) ;
#5689=CARTESIAN_POINT ( 'NONE',  ( -74.10069187148681635, -293.4294371709647749, -204.1109707557360480 ) ) ;
#5690=CARTESIAN_POINT ( 'NONE',  ( 19.06348109387202427, -291.5292691793140420, -218.6721075036340380 ) ) ;
#5691=CARTESIAN_POINT ( 'NONE',  ( -24.54357031718447502, -273.2781073344021934, -198.2009966241897132 ) ) ;
#5692=CARTESIAN_POINT ( 'NONE',  ( 23.08641555477721852, -293.5378020024226657, -317.9401603438001871 ) ) ;
#5693=CARTESIAN_POINT ( 'NONE',  ( -48.18191685322902629, -287.6723078097360258, -343.3043088307907738 ) ) ;
#5694=CARTESIAN_POINT ( 'NONE',  ( 35.91385957964418196, -291.6545582059508206, -259.7971705390189072 ) ) ;
#5695=CARTESIAN_POINT ( 'NONE',  ( -98.43270965734657807, -291.1952627253893979, -311.0659171504086089 ) ) ;
#5697=CARTESIAN_POINT ( 'NONE',  ( -111.8241535989361921, -292.4338905136488052, -279.5842747142044118 ) ) ;
#5698=CARTESIAN_POINT ( 'NONE',  ( -52.98236629898809724, -289.8520940846919984, -196.7865093995712868 ) ) ;
#5699=CARTESIAN_POINT ( 'NONE',  ( 18.04964310311467912, -294.8462736330813527, -219.7774443756317169 ) ) ;
#5700=CARTESIAN_POINT ( 'NONE',  ( -49.47226760900633735, -286.8350919067108293, -198.0857872087619569 ) ) ;
#5701=CARTESIAN_POINT ( 'NONE',  ( 37.87700061916662264, -295.5513509968073436, -270.2857543416536714 ) ) ;
#5703=CARTESIAN_POINT ( 'NONE',  ( 36.59983589094233736, -277.3463855304444223, -255.8333495072104142 ) ) ;
#5704=CARTESIAN_POINT ( 'NONE',  ( -99.88304356740698609, -295.1557659750702101, -315.0908592908771197 ) ) ;
#5705=CARTESIAN_POINT ( 'NONE',  ( -46.27922519421891678, -272.1770656965683770, -196.8893910525438571 ) ) ;
#5706=CARTESIAN_POINT ( 'NONE',  ( -105.7560830810136565, -277.0185169427158485, -241.0219564342388594 ) ) ;
#5707=CARTESIAN_POINT ( 'NONE',  ( -62.17841503435602135, -274.9268970051939505, -201.2939905102009561 ) ) ;
#5709=CARTESIAN_POINT ( 'NONE',  ( 19.60893185760472690, -273.4299810725545399, -219.3399212466285633 ) ) ;
#5710=CARTESIAN_POINT ( 'NONE',  ( -78.26244330558120055, -297.0394230667206443, -331.5852901726725577 ) ) ;
#5713=CARTESIAN_POINT ( 'NONE',  ( -110.2121295165967041, -297.4480078387508684, -263.2942035712040365 ) ) ;
#5715=CARTESIAN_POINT ( 'NONE',  ( 35.11680370657025918, -285.3050716513362204, -249.4832955014770448 ) ) ;
#5716=CARTESIAN_POINT ( 'NONE',  ( -91.12109969885604244, -273.0941141046508278, -220.9789011326918171 ) ) ;
#5717=CARTESIAN_POINT ( 'NONE',  ( 0.2837910275786243997, -286.5389369130856494, -203.1648049954682449 ) ) ;
#5718=CARTESIAN_POINT ( 'NONE',  ( -12.23463671024023469, -288.4010994954074931, -343.1863322452018679 ) ) ;
#5719=CARTESIAN_POINT ( 'NONE',  ( -100.2411356184922653, -297.9733513908078066, -311.9532453549978754 ) ) ;
#5720=CARTESIAN_POINT ( 'NONE',  ( -15.07091183603833606, -292.7630281916104309, -341.8581856210194019 ) ) ;
#5721=CARTESIAN_POINT ( 'NONE',  ( 39.25156628236135248, -280.6724415336311154, -264.2267589533992123 ) ) ;
#5722=CARTESIAN_POINT ( 'NONE',  ( -114.2704648735229114, -288.0523547857347353, -270.3284710469133074 ) ) ;
#5724=CARTESIAN_POINT ( 'NONE',  ( -71.37040974471354104, -288.3068889793354970, -335.4074447466838933 ) ) ;
#5725=DIRECTION ( 'NONE',  ( 1.000000000000000000, 0.000000000000000000, 0.000000000000000000 ) ) ;
#5726=CARTESIAN_POINT ( 'NONE',  ( -4.951124841408945265, -286.6255172697171361, -338.0061568715209432 ) ) ;
#5727=CARTESIAN_POINT ( 'NONE',  ( -58.14964194610149661, -299.3788856748544163, -199.5552568497616335 ) ) ;
#5728=CARTESIAN_POINT ( 'NONE',  ( -40.99849454269833871, -281.4322804819817065, -194.0248019828148074 ) ) ;
#5729=CARTESIAN_POINT ( 'NONE',  ( -88.47333119696713766, -295.3601341879847269, -214.9373793898434712 ) ) ;
#5730=CARTESIAN_POINT ( 'NONE',  ( 32.95944695222735277, -281.8120796101092651, -290.0270458577659838 ) ) ;
#5731=CARTESIAN_POINT ( 'NONE',  ( -103.1144836723647842, -296.1960357467776817, -310.3978629717748845 ) ) ;
#5732=CARTESIAN_POINT ( 'NONE',  ( -40.56751366323234009, -299.5310126236279302, -196.7257506761647221 ) ) ;
#5734=CARTESIAN_POINT ( 'NONE',  ( 19.53237840017119709, -282.8745502570830581, -221.4504962905907064 ) ) ;
#5735=CARTESIAN_POINT ( 'NONE',  ( -94.84666163405515249, -272.1114295819882045, -224.8923872227141771 ) ) ;
#5738=CARTESIAN_POINT ( 'NONE',  ( -33.38436722844436133, -284.9820075898539926, -344.9138041418873968 ) ) ;
#5740=CARTESIAN_POINT ( 'NONE',  ( -111.2586520408596868, -282.4809262143061233, -234.7283546768995564 ) ) ;
#5741=CARTESIAN_POINT ( 'NONE',  ( -14.64716392923073940, -275.9626250096894182, -343.8274285040680525 ) ) ;
#5742=CARTESIAN_POINT ( 'NONE',  ( 24.84898362760958435, -292.8573758270937901, -232.0379498484602152 ) ) ;
#5743=CARTESIAN_POINT ( 'NONE',  ( -100.9903167747113315, -285.5672894443194991, -307.5035647269911010 ) ) ;
#5744=CARTESIAN_POINT ( 'NONE',  ( 36.17321144128678867, -277.0604677543070125, -263.3244181971031139 ) ) ;
#5745=CARTESIAN_POINT ( 'NONE',  ( -81.20832872910371236, -285.0603891834516048, -332.9900459075452090 ) ) ;
#5746=CARTESIAN_POINT ( 'NONE',  ( -26.70029019215288812, -281.7088385231738243, -343.0342547923207803 ) ) ;
#5747=CARTESIAN_POINT ( 'NONE',  ( -21.80428313474043733, -282.2513104832187878, -196.9348965000683904 ) ) ;
#5748=CARTESIAN_POINT ( 'NONE',  ( -10.34960310997828437, -274.5613809887775005, -198.1904111299019462 ) ) ;
#5749=CARTESIAN_POINT ( 'NONE',  ( 38.73541738247091359, -275.5383055247751258, -282.5814994750116966 ) ) ;
#5750=CARTESIAN_POINT ( 'NONE',  ( -91.43719314619438876, -297.7492393989813309, -321.5723146638374033 ) ) ;
#5753=CARTESIAN_POINT ( 'NONE',  ( -93.74808097261622208, -293.9941146111855801, -320.9633141822506559 ) ) ;
#5755=CARTESIAN_POINT ( 'NONE',  ( 28.08282000434283532, -275.5017722808886447, -302.9962290752318950 ) ) ;
#5756=CARTESIAN_POINT ( 'NONE',  ( -11.27568569241208785, -296.2388330997546291, -342.1337832458915500 ) ) ;
#5757=CARTESIAN_POINT ( 'NONE',  ( 35.99405036289560655, -295.0385126541833074, -292.6740819260873536 ) ) ;
#5758=CARTESIAN_POINT ( 'NONE',  ( -89.93181438835244990, -291.7971315196407431, -323.5993402230953961 ) ) ;
#5760=CARTESIAN_POINT ( 'NONE',  ( -95.90326972664253447, -275.9099979619981013, -316.9709816389230355 ) ) ;
#5761=CARTESIAN_POINT ( 'NONE',  ( -111.8328312978207038, -280.4683440362146598, -270.6679211818018302 ) ) ;
#5762=CARTESIAN_POINT ( 'NONE',  ( -110.6906650645110517, -294.7962657508849702, -257.6629471649252423 ) ) ;
#5763=CARTESIAN_POINT ( 'NONE',  ( -3.424198218548725414, -284.4696627206279231, -338.1244018102202631 ) ) ;
#5764=CARTESIAN_POINT ( 'NONE',  ( -107.6474953668672043, -283.7482173354496808, -249.4168986826251455 ) ) ;
#5765=CARTESIAN_POINT ( 'NONE',  ( 199.0957512885324832, 283.1197628812451512, -111.3260668811493588 ) ) ;
#5767=CARTESIAN_POINT ( 'NONE',  ( -93.26856050096415629, -284.8854125089400782, -223.4114238867873041 ) ) ;
#5769=CARTESIAN_POINT ( 'NONE',  ( 21.72380857055593140, -281.9715754237286092, -221.4452903483682462 ) ) ;
#5770=CARTESIAN_POINT ( 'NONE',  ( -93.61754808071229661, -284.0590748799286303, -218.3118881252798360 ) ) ;
#5771=CARTESIAN_POINT ( 'NONE',  ( -59.24650316674426875, -280.7165931589534580, -196.7880263238149325 ) ) ;
#5772=CARTESIAN_POINT ( 'NONE',  ( -34.29918604931301473, -278.5346647396338540, -346.6071071368523917 ) ) ;
#5773=CARTESIAN_POINT ( 'NONE',  ( -38.17713146789083822, -280.6933493872815006, -193.4675887256294970 ) ) ;
#5774=CARTESIAN_POINT ( 'NONE',  ( -105.5795714935544112, -270.2666405000204009, -254.7536222014695397 ) ) ;
#5775=CARTESIAN_POINT ( 'NONE',  ( 154.7580071528325334, 206.6321147285761128, -217.3817845441456313 ) ) ;
#5776=CARTESIAN_POINT ( 'NONE',  ( -66.55167080091212028, -275.6688505014986390, -201.4640495272424516 ) ) ;
#5777=CARTESIAN_POINT ( 'NONE',  ( -78.43836082823335687, -208.2269359979451906, -356.9560842802424077 ) ) ;
#5778=CARTESIAN_POINT ( 'NONE',  ( -66.69376542947502173, -277.6858607376447026, -201.7155263566453129 ) ) ;
#5779=CARTESIAN_POINT ( 'NONE',  ( -22.41507573805834497, -294.0007421626194173, -195.8013359161006974 ) ) ;
#5780=CARTESIAN_POINT ( 'NONE',  ( -94.85877176721795934, -295.2654161726230200, -315.4796190505793447 ) ) ;
#5781=CARTESIAN_POINT ( 'NONE',  ( -82.82131920756381760, -289.1634266546830077, -332.4186006212438542 ) ) ;
#5783=CARTESIAN_POINT ( 'NONE',  ( -8.626442225939685571, -293.2585141297187192, -341.2270487516418598 ) ) ;
#5784=CARTESIAN_POINT ( 'NONE',  ( -35.89760245871006106, -284.4704337206260902, -196.5752453565859810 ) ) ;
#5785=CARTESIAN_POINT ( 'NONE',  ( -14.48827413641327411, -294.2120065649813228, -199.7311923199909245 ) ) ;
#5786=CARTESIAN_POINT ( 'NONE',  ( 13.63298984349051679, -285.2614928419181410, -217.0714452925102762 ) ) ;
#5787=CARTESIAN_POINT ( 'NONE',  ( -78.64001308422193404, -284.9366157854417452, -331.1533282075482134 ) ) ;
#5789=CARTESIAN_POINT ( 'NONE',  ( -105.7997235108398115, -291.9432418997286049, -235.5117711052858169 ) ) ;
#5790=CARTESIAN_POINT ( 'NONE',  ( 34.54712625196881959, -282.2172714786458982, -283.4690862023936120 ) ) ;
#5791=CARTESIAN_POINT ( 'NONE',  ( 39.25952395753014201, -292.3106952854265046, -267.4669932054571859 ) ) ;
#5792=CARTESIAN_POINT ( 'NONE',  ( -20.52177345904916450, -289.6444253021045370, -345.3906608123761544 ) ) ;
#5793=CARTESIAN_POINT ( 'NONE',  ( -113.0716152599298852, -290.8735520198528093, -284.0188298889467546 ) ) ;
#5794=CARTESIAN_POINT ( 'NONE',  ( 29.96094601394658241, -287.3378921394774466, -241.9573737839068031 ) ) ;
#5797=CARTESIAN_POINT ( 'NONE',  ( -111.9273842800553496, -298.5817978326583102, -257.0464192749748804 ) ) ;
#5798=CARTESIAN_POINT ( 'NONE',  ( -36.53018448292221620, -296.7469447127292597, -193.8544420277347911 ) ) ;
#5799=CARTESIAN_POINT ( 'NONE',  ( 30.24322696499087826, -280.2337310311822307, -242.1532099189585665 ) ) ;
#5801=CARTESIAN_POINT ( 'NONE',  ( -3.457967597231253354, -297.8145302279941120, -193.4666757322721935 ) ) ;
#5802=CARTESIAN_POINT ( 'NONE',  ( -78.35149933882429707, -294.0945031370173410, -331.6510593981409443 ) ) ;
#5803=CARTESIAN_POINT ( 'NONE',  ( 34.22771967064979037, -277.5579536409021557, -289.2235718302286500 ) ) ;
#5804=CARTESIAN_POINT ( 'NONE',  ( -93.83869082295066733, -271.3655235580656608, -222.1859689139305090 ) ) ;
#5805=CARTESIAN_POINT ( 'NONE',  ( -4.143403643652741053, -295.8094317599079659, -335.8351325582482900 ) ) ;
#5806=CARTESIAN_POINT ( 'NONE',  ( -106.2731608860714232, -297.2990385937704900, -295.4638574129397739 ) ) ;
#5808=CARTESIAN_POINT ( 'NONE',  ( -27.82730623010683857, -296.5335250004055752, -346.0175395129002140 ) ) ;
#5809=CARTESIAN_POINT ( 'NONE',  ( -40.34097257410225268, -296.0145062489132215, -195.2034221697184648 ) ) ;
#5810=CARTESIAN_POINT ( 'NONE',  ( -32.15832675795920892, -292.7706406046042957, -197.4305446049828845 ) ) ;
#5811=CARTESIAN_POINT ( 'NONE',  ( -96.81760244974110208, -274.0096978011514466, -221.6910622589487048 ) ) ;
#5812=CARTESIAN_POINT ( 'NONE',  ( -110.8329621990606455, -289.1881273338095184, -265.6801956808976115 ) ) ;
#5813=CARTESIAN_POINT ( 'NONE',  ( 121.3395553409046528, -299.5541904835127980, -195.3611179825600175 ) ) ;
#5814=CARTESIAN_POINT ( 'NONE',  ( -70.11126143934319543, -274.1243107896996776, -200.7357772458493912 ) ) ;
#5815=CARTESIAN_POINT ( 'NONE',  ( -97.19827691613841125, -296.3024119178330693, -312.1854853061793165 ) ) ;
#5816=CARTESIAN_POINT ( 'NONE',  ( -6.918054506879156129, -282.4292894281523445, -201.4065367525154500 ) ) ;
#5817=CARTESIAN_POINT ( 'NONE',  ( 31.58450669542373745, -279.8069066511179130, -237.0356233251795572 ) ) ;
#5818=CARTESIAN_POINT ( 'NONE',  ( -4.046500103412615346, -275.9731549710980403, -339.6918461529121487 ) ) ;
#5819=CARTESIAN_POINT ( 'NONE',  ( 34.57945288242659387, -279.6293744593503448, -245.0282495480993532 ) ) ;
#5820=CARTESIAN_POINT ( 'NONE',  ( -3.735904834450111345, -280.6097109895972039, -337.6114148401288730 ) ) ;
#5822=CARTESIAN_POINT ( 'NONE',  ( -63.49933604404081677, -272.2792023331933819, -201.5641396797239793 ) ) ;
#5823=CARTESIAN_POINT ( 'NONE',  ( -112.0611173911752303, -280.6427900891960689, -263.3147681650081040 ) ) ;
#5827=CARTESIAN_POINT ( 'NONE',  ( 96.97712259441328797, -297.9515605777340284, -194.4139984393089549 ) ) ;
#5828=CARTESIAN_POINT ( 'NONE',  ( 22.68073234451026465, -290.9516883036625927, -224.7798666402447054 ) ) ;
#5829=CARTESIAN_POINT ( 'NONE',  ( -70.89771341143497807, -291.6215903590082235, -201.0574819125283454 ) ) ;
#5830=CARTESIAN_POINT ( 'NONE',  ( -37.10650145541197986, -279.0493349585280498, -345.5401692336875499 ) ) ;
#5831=CARTESIAN_POINT ( 'NONE',  ( -26.98959127535904301, -272.1834772614915892, -196.0266959755703340 ) ) ;
#5833=CARTESIAN_POINT ( 'NONE',  ( 29.80881533814829609, -283.9273444942072047, -305.0039017601280307 ) ) ;
#5835=CARTESIAN_POINT ( 'NONE',  ( 18.42569466378405352, -286.2509335325852362, -320.5297634117886787 ) ) ;
#5837=CARTESIAN_POINT ( 'NONE',  ( -18.13127116356609037, -293.5938725927802011, -341.1995956816894022 ) ) ;
#5838=CARTESIAN_POINT ( 'NONE',  ( 34.22629246734285147, -285.4354960076999532, -250.6408766576362837 ) ) ;
#5840=CARTESIAN_POINT ( 'NONE',  ( 32.43722319485794259, -291.9115183176212440, -297.9967698098740243 ) ) ;
#5841=CARTESIAN_POINT ( 'NONE',  ( -47.18625929612417735, -281.6549466116007920, -346.0300839222187506 ) ) ;
#5842=CARTESIAN_POINT ( 'NONE',  ( -43.84163656708467016, -281.5689117503197849, -196.7971289869299198 ) ) ;
#5843=CARTESIAN_POINT ( 'NONE',  ( -107.5682853823894902, -286.1508145804614855, -239.6304621266478989 ) ) ;
#5844=CARTESIAN_POINT ( 'NONE',  ( 37.14769176420034569, -279.9822424444057560, -285.3712649446937348 ) ) ;
#5845=CARTESIAN_POINT ( 'NONE',  ( 34.52168923811392176, -287.7214239878546209, -283.1928469698248705 ) ) ;
#5846=CARTESIAN_POINT ( 'NONE',  ( -101.3330633903045737, -280.4711055189549711, -234.0227038217660152 ) ) ;
#5847=CARTESIAN_POINT ( 'NONE',  ( -102.3039594605032931, -279.8129579991354490, -236.5980959320195609 ) ) ;
#5849=CARTESIAN_POINT ( 'NONE',  ( -18.61567453809499639, -288.2719225488984875, -197.3158088079621564 ) ) ;
#5851=CARTESIAN_POINT ( 'NONE',  ( -9.108184373951473844, -298.2298170564640714, -193.3618857822629593 ) ) ;
#5852=CARTESIAN_POINT ( 'NONE',  ( -99.68690915034417799, -293.0898461000305133, -229.2193848998570900 ) ) ;
#5854=CARTESIAN_POINT ( 'NONE',  ( -115.3430155898818299, -299.2662352645559167, -252.5904736702033517 ) ) ;
#5856=CARTESIAN_POINT ( 'NONE',  ( -3.362946426965163216, -272.4995135873649588, -203.2984767044623027 ) ) ;
#5857=CARTESIAN_POINT ( 'NONE',  ( -25.05707791679039431, -293.2980154564169197, -345.6178675202841077 ) ) ;
#5858=CARTESIAN_POINT ( 'NONE',  ( -72.87132862955478174, -297.0754529053523925, -206.5204260980227673 ) ) ;
#5859=CARTESIAN_POINT ( 'NONE',  ( 22.53624336083535695, -289.6671109006661595, -313.3185345365367311 ) ) ;
#5861=CARTESIAN_POINT ( 'NONE',  ( 7.742074953156449446, -282.4370734769851765, -211.5985254147447279 ) ) ;
#5862=CARTESIAN_POINT ( 'NONE',  ( -77.80883846843350682, -291.0092274865546642, -335.2380841106740945 ) ) ;
#5863=CARTESIAN_POINT ( 'NONE',  ( -113.1796150786164503, -291.9992784467313527, -259.8776398959319636 ) ) ;
#5864=CARTESIAN_POINT ( 'NONE',  ( -35.92042454816522934, -288.0701400924353948, -195.3745816696648490 ) ) ;
#5865=CARTESIAN_POINT ( 'NONE',  ( -103.4126861797397368, -279.2356109739591261, -230.7147441718757364 ) ) ;
#5866=CARTESIAN_POINT ( 'NONE',  ( -1.412850710840422686, -292.6594512925507274, -336.8470096827380758 ) ) ;
#5867=CARTESIAN_POINT ( 'NONE',  ( 21.06748726530683413, -280.7080599864149235, -220.1677005407295837 ) ) ;
#5868=CARTESIAN_POINT ( 'NONE',  ( 32.43070515813587917, -277.7464761711309507, -295.8617034362296181 ) ) ;
#5870=CARTESIAN_POINT ( 'NONE',  ( -110.4542110544635705, -298.8376638359844719, -287.0812184334320705 ) ) ;
#5871=CARTESIAN_POINT ( 'NONE',  ( 26.09706842815266725, -273.2346856866873850, -228.5341331829797298 ) ) ;
#5873=CARTESIAN_POINT ( 'NONE',  ( 28.20350686436677279, -281.4981943882946780, -302.7530596194822579 ) ) ;
#5874=CARTESIAN_POINT ( 'NONE',  ( -54.02971886978359350, -278.4667498916023192, -345.1785584520411021 ) ) ;
#5875=CARTESIAN_POINT ( 'NONE',  ( -109.6177798865284672, -274.0454297395746721, -256.7689657923062327 ) ) ;
#5876=CARTESIAN_POINT ( 'NONE',  ( -113.9161884942815277, -283.6875017427759076, -264.2549829255597160 ) ) ;
#5877=CARTESIAN_POINT ( 'NONE',  ( -91.51597573476546188, -293.0276038846615734, -219.9129978082602292 ) ) ;
#5878=CARTESIAN_POINT ( 'NONE',  ( -49.61072543368067045, -275.4984689368752129, -195.1020761104337851 ) ) ;
#5879=CARTESIAN_POINT ( 'NONE',  ( -106.4052874089918106, -274.2920130612158118, -237.4442654095895193 ) ) ;
#5881=CARTESIAN_POINT ( 'NONE',  ( 20.02114368815130163, -276.0225754703945995, -315.5310451171347381 ) ) ;
#5882=CARTESIAN_POINT ( 'NONE',  ( -104.3999815358387906, -298.1117102159607839, -303.6928239167373818 ) ) ;
#5883=CARTESIAN_POINT ( 'NONE',  ( -110.5180462890020578, -282.3496828256400590, -286.0825592521257477 ) ) ;
#5884=CARTESIAN_POINT ( 'NONE',  ( -61.67787143112253290, -291.4112298820096498, -197.2741960514575226 ) ) ;
#5885=CARTESIAN_POINT ( 'NONE',  ( 31.70568001355369958, -273.1989561112062574, -241.8649895559216532 ) ) ;
#5886=CARTESIAN_POINT ( 'NONE',  ( 19.04611703627797326, -289.8562758818808902, -321.6334080570705396 ) ) ;
#5887=CARTESIAN_POINT ( 'NONE',  ( -109.9309595453163411, -289.3366708692947213, -280.6994902012481816 ) ) ;
#5889=CARTESIAN_POINT ( 'NONE',  ( -111.7393844530081850, -289.3464831604720189, -252.9372589780034559 ) ) ;
#5890=CARTESIAN_POINT ( 'NONE',  ( -87.94218381655042549, -290.9877484713275066, -217.6445101868062579 ) ) ;
#5892=CARTESIAN_POINT ( 'NONE',  ( 39.04545297181316954, -288.5390541985246955, -262.9733086454263571 ) ) ;
#5893=CARTESIAN_POINT ( 'NONE',  ( -93.10909541348289054, -279.5553360123302014, -223.2028849580876511 ) ) ;
#5894=CARTESIAN_POINT ( 'NONE',  ( -81.70414139475033721, -294.5605846921813509, -332.9836907621987621 ) ) ;
#5895=CARTESIAN_POINT ( 'NONE',  ( -66.52986655384275139, -284.0759175334835618, -341.5185463276025075 ) ) ;
#5896=CARTESIAN_POINT ( 'NONE',  ( -104.3965106526863735, -284.3934798537279676, -308.2764333612271912 ) ) ;
#5898=CARTESIAN_POINT ( 'NONE',  ( -16.12230466580236765, -283.1033664215912609, -340.2311741076330236 ) ) ;
#5899=CARTESIAN_POINT ( 'NONE',  ( 121.5737172192837647, 149.6818241901583519, -263.5908535195870854 ) ) ;
#5900=CARTESIAN_POINT ( 'NONE',  ( 200.5336724191271287, 293.3464715333668664, -82.97196496506106200 ) ) ;
#5901=CARTESIAN_POINT ( 'NONE',  ( 201.2091503359040416, 293.0224724744892910, -53.99999999998772893 ) ) ;
#5902=CARTESIAN_POINT ( 'NONE',  ( 20.14300298717034465, -275.3865259312892704, -315.6373465373062004 ) ) ;
#5903=CARTESIAN_POINT ( 'NONE',  ( 25.54805180592470393, -273.9553379912273385, -232.5917511904098660 ) ) ;
#5904=CARTESIAN_POINT ( 'NONE',  ( -53.28262368708350039, -294.7588242118001176, -345.6845620427292261 ) ) ;
#5905=CARTESIAN_POINT ( 'NONE',  ( -37.97421885051181079, -140.6615534827124065, -361.4716249991672612 ) ) ;
#5906=CARTESIAN_POINT ( 'NONE',  ( 28.08953652310458793, -273.7149588171571963, -230.6106996128995377 ) ) ;
#5907=CARTESIAN_POINT ( 'NONE',  ( -52.91698336635150213, -299.7109788148400185, -197.7254607410615108 ) ) ;
#5908=CARTESIAN_POINT ( 'NONE',  ( -41.62458576998787407, -293.0767583622085226, -197.1271626203962626 ) ) ;
#5910=CARTESIAN_POINT ( 'NONE',  ( -110.5717227983794970, -297.2026739782708091, -293.4308178788953114 ) ) ;
#5911=CARTESIAN_POINT ( 'NONE',  ( -3.332142614293172933, -289.0830067836944863, -335.0804222139351509 ) ) ;
#5912=CARTESIAN_POINT ( 'NONE',  ( -113.6157304054386401, -297.4714964996462641, -261.0642838139588662 ) ) ;
#5913=CARTESIAN_POINT ( 'NONE',  ( -95.53084320546444985, -296.3639744853335856, -320.6955051478072392 ) ) ;
#5914=CARTESIAN_POINT ( 'NONE',  ( 29.85491414142531497, -293.3343197721284241, -241.7078647926716712 ) ) ;
#5916=CARTESIAN_POINT ( 'NONE',  ( 38.19072379062034628, -277.4462914734339734, -268.3197625022576176 ) ) ;
#5919=CARTESIAN_POINT ( 'NONE',  ( 6.154632182364051296, -280.1330478315038022, -206.8977744003737200 ) ) ;
#5920=CARTESIAN_POINT ( 'NONE',  ( -0.4380277963570491928, -275.4969204518833976, -207.0888539788068385 ) ) ;
#5921=CARTESIAN_POINT ( 'NONE',  ( -21.58705511561383261, -276.0116050854931018, -196.0256273214094449 ) ) ;
#5922=CARTESIAN_POINT ( 'NONE',  ( -95.79486251683916009, -275.9200123858412894, -317.9379783407196101 ) ) ;
#5923=CARTESIAN_POINT ( 'NONE',  ( -37.15767395580831334, -298.7059386433933241, -197.2563104522588162 ) ) ;
#5924=CARTESIAN_POINT ( 'NONE',  ( -66.30160080640023068, -294.0136355706548557, -338.0124230023276368 ) ) ;
#5926=CARTESIAN_POINT ( 'NONE',  ( -94.91990408976175786, -279.7364432972652821, -219.3289973929232133 ) ) ;
#5927=CARTESIAN_POINT ( 'NONE',  ( -21.65095256143696290, -277.0121800002983150, -341.7068723450335028 ) ) ;
#5928=CARTESIAN_POINT ( 'NONE',  ( 2.498593096772880884, -285.2593198525837579, -205.0461173462174713 ) ) ;
#5929=CARTESIAN_POINT ( 'NONE',  ( -77.25115969597118237, -299.5185044677735959, -206.6644660885268934 ) ) ;
#5930=CARTESIAN_POINT ( 'NONE',  ( 82.66436015057398379, -298.3400917633185827, -197.5716692144941362 ) ) ;
#5931=CARTESIAN_POINT ( 'NONE',  ( 35.61206425292357380, -286.8301847085243708, -276.5050500214535418 ) ) ;
#5932=CARTESIAN_POINT ( 'NONE',  ( -21.96225826316446827, -278.4916138296314330, -197.9107010581973896 ) ) ;
#5933=CARTESIAN_POINT ( 'NONE',  ( -102.6706824402684077, -277.5852116543040893, -236.3755129093389371 ) ) ;
#5934=CARTESIAN_POINT ( 'NONE',  ( -110.1332356122260592, -282.4296763044688987, -286.0007928923134273 ) ) ;
#5935=CARTESIAN_POINT ( 'NONE',  ( -57.90628777537927618, -287.7868294318164430, -198.1823433619638308 ) ) ;
#5936=CARTESIAN_POINT ( 'NONE',  ( 18.62106700892852729, -277.4288014158954070, -317.8511085088505297 ) ) ;
#5938=CARTESIAN_POINT ( 'NONE',  ( -95.91793325527721947, -293.1963925842221101, -223.5228263150655152 ) ) ;
#5939=CARTESIAN_POINT ( 'NONE',  ( -20.37447151732715867, -275.0771153282910291, -344.4832379296491354 ) ) ;
#5940=CARTESIAN_POINT ( 'NONE',  ( 7.386746795288989809, -275.3321910576300979, -212.5401987261823251 ) ) ;
#5941=CARTESIAN_POINT ( 'NONE',  ( 36.62615812048505859, -283.7245304329682085, -283.8037696818990412 ) ) ;
#5943=CARTESIAN_POINT ( 'NONE',  ( 38.16662097048998703, -289.5227957866670181, -274.3225937122457481 ) ) ;
#5944=CARTESIAN_POINT ( 'NONE',  ( -9.808272363124412863, -292.6925230793752348, -340.1792265857679922 ) ) ;
#5946=CARTESIAN_POINT ( 'NONE',  ( 31.58660314724305707, -273.8992607641877726, -244.8634223043338238 ) ) ;
#5947=CARTESIAN_POINT ( 'NONE',  ( 35.93699067301943728, -291.5366098952956690, -258.4029661927262964 ) ) ;
#5948=CARTESIAN_POINT ( 'NONE',  ( 207.9738562182569979, 296.4636489450776367, -53.99999999999996447 ) ) ;
#5950=CARTESIAN_POINT ( 'NONE',  ( -81.51314198400530131, -289.9429385321560062, -208.1390039435764834 ) ) ;
#5951=CARTESIAN_POINT ( 'NONE',  ( 36.15847101141952891, -286.0365693578910964, -289.6406111922293007 ) ) ;
#5952=CARTESIAN_POINT ( 'NONE',  ( -90.09784014928001739, -286.7140129219131950, -218.9833481387612721 ) ) ;
#5953=CARTESIAN_POINT ( 'NONE',  ( -98.24714543452139992, -285.9164405738245023, -229.8255970284060936 ) ) ;
#5954=CARTESIAN_POINT ( 'NONE',  ( -112.7440084987078279, -292.5208747485262961, -271.2353873984615689 ) ) ;
#5955=CARTESIAN_POINT ( 'NONE',  ( 33.38267531793234610, -273.2891149986369328, -243.7645596713856264 ) ) ;
#5956=CARTESIAN_POINT ( 'NONE',  ( 3.493883597693932419, -276.8526407094437900, -335.6787470154824291 ) ) ;
#5957=CARTESIAN_POINT ( 'NONE',  ( -111.5067524685816664, -288.8170458532259204, -255.8418640012977221 ) ) ;
#5958=CARTESIAN_POINT ( 'NONE',  ( 16.95522598451886154, -276.3046930662062550, -325.0326752986218821 ) ) ;
#5959=CARTESIAN_POINT ( 'NONE',  ( -98.51724811578361596, -297.9487570645957817, -313.1325936664433129 ) ) ;
#5962=CARTESIAN_POINT ( 'NONE',  ( -97.75182001462053449, -283.8164844320434099, -228.4836425946084830 ) ) ;
#5963=CARTESIAN_POINT ( 'NONE',  ( 5.074684711517985392, -278.6254773587518798, -208.5076545095119513 ) ) ;
#5965=CARTESIAN_POINT ( 'NONE',  ( 37.49854503773154590, -274.2199196149044838, -285.2488800054418334 ) ) ;
#5966=CARTESIAN_POINT ( 'NONE',  ( -16.35953576138010845, -276.1224003591457290, -340.4402045645200019 ) ) ;
#5967=CARTESIAN_POINT ( 'NONE',  ( 29.02732323551024507, -295.5030334922710722, -302.5079214175981406 ) ) ;
#5968=CARTESIAN_POINT ( 'NONE',  ( 6.020844782299992204, -279.5458182110612597, -207.1062192951671079 ) ) ;
#5969=CARTESIAN_POINT ( 'NONE',  ( 17.26398336829361568, -295.1894305148285298, -319.1819527188986285 ) ) ;
#5971=CARTESIAN_POINT ( 'NONE',  ( -65.40690521778019217, -296.7266210566795053, -341.5485748630854914 ) ) ;
#5972=CARTESIAN_POINT ( 'NONE',  ( -109.9063062625910874, -272.3263847655838390, -262.2084850772610025 ) ) ;
#5973=CARTESIAN_POINT ( 'NONE',  ( -111.6860408655634842, -292.6843288238685545, -260.0795071766720525 ) ) ;
#5974=CARTESIAN_POINT ( 'NONE',  ( -104.0415186784035200, -285.2201666703302863, -231.7825687038794626 ) ) ;
#5975=CARTESIAN_POINT ( 'NONE',  ( -10.75844407506960110, -272.5346119203353510, -199.3571753994172582 ) ) ;
#5976=CARTESIAN_POINT ( 'NONE',  ( 0.2856448581120792918, -286.3722837850887117, -203.1658430544205487 ) ) ;
#5977=CARTESIAN_POINT ( 'NONE',  ( -102.2543164025909732, -281.0256360975375287, -233.5073658163543939 ) ) ;
#5979=CARTESIAN_POINT ( 'NONE',  ( -2.062546817588094328, -285.5898173759450742, -206.1264164768845433 ) ) ;
#5980=CARTESIAN_POINT ( 'NONE',  ( -51.33771324277528691, -287.2309533507367973, -344.0436278660727680 ) ) ;
#5981=CARTESIAN_POINT ( 'NONE',  ( -110.2140734402150315, -271.0703965937372004, -283.6296548450457635 ) ) ;
#5982=CARTESIAN_POINT ( 'NONE',  ( -37.27452594576047318, -285.5606305738032802, -197.2871612464168720 ) ) ;
#5983=CARTESIAN_POINT ( 'NONE',  ( -34.47571799833898609, -283.9581991348520660, -347.0723059537602921 ) ) ;
#5984=CARTESIAN_POINT ( 'NONE',  ( -73.31281617031996234, -290.6457803915457703, -202.5310819535010012 ) ) ;
#5985=CARTESIAN_POINT ( 'NONE',  ( -113.4320613315310311, -280.1006389850841174, -274.4473565415793246 ) ) ;
#5986=CARTESIAN_POINT ( 'NONE',  ( -110.0860468285261504, -280.1692626991464294, -246.4956362764479820 ) ) ;
#5987=CARTESIAN_POINT ( 'NONE',  ( 13.33662947264594933, -280.6182732636815444, -217.7482428526018339 ) ) ;
#5988=CARTESIAN_POINT ( 'NONE',  ( 36.68530665664987822, -277.7109644365514782, -282.7172801949819814 ) ) ;
#5989=CARTESIAN_POINT ( 'NONE',  ( -95.58149718973983511, -295.8717068608051477, -320.7310101624807430 ) ) ;
#5990=CARTESIAN_POINT ( 'NONE',  ( -99.49386711827017393, -288.0108085991494704, -311.7239071073950072 ) ) ;
#5991=CARTESIAN_POINT ( 'NONE',  ( -108.1305717749185646, -295.7236991369195493, -251.2559772775269096 ) ) ;
#5993=CARTESIAN_POINT ( 'NONE',  ( 22.17568282459027529, -284.0881698145445853, -315.0923159870245627 ) ) ;
#5994=CARTESIAN_POINT ( 'NONE',  ( -68.53022372016609154, -295.1402955790632632, -336.4003295392051314 ) ) ;
#5995=CARTESIAN_POINT ( 'NONE',  ( 37.75640112553596595, -294.4357669153371262, -254.7479280267220929 ) ) ;
#5996=CARTESIAN_POINT ( 'NONE',  ( -7.203884436192401708, -283.2974898235943897, -336.9751873970264455 ) ) ;
#5997=CARTESIAN_POINT ( 'NONE',  ( -27.01626463977208203, -273.2389828234658466, -194.2407382155091398 ) ) ;
#5998=CARTESIAN_POINT ( 'NONE',  ( -110.6821137467765084, -290.9106764461627108, -293.6541972034444257 ) ) ;
#5999=CARTESIAN_POINT ( 'NONE',  ( -23.98007752674210380, -284.3605149886851677, -195.7304757717481607 ) ) ;
#6000=CARTESIAN_POINT ( 'NONE',  ( -94.69838580893468816, -291.5820447233759865, -219.0195665913088590 ) ) ;
#6001=CARTESIAN_POINT ( 'NONE',  ( 23.54934965867307639, -287.3253151340538238, -229.9661372154001242 ) ) ;
#6004=CARTESIAN_POINT ( 'NONE',  ( -88.43586288902518788, -229.5806346048500473, -344.3981502665915286 ) ) ;
#6005=CARTESIAN_POINT ( 'NONE',  ( -73.92639662551032131, -285.0487258973328721, -337.3847428240234763 ) ) ;
#6006=CARTESIAN_POINT ( 'NONE',  ( 35.78497577281001440, -290.8380690714490129, -253.7030783399848985 ) ) ;
#6007=EDGE_LOOP ( 'NONE', ( #87173, #92982 ) ) ;
#6008=CARTESIAN_POINT ( 'NONE',  ( -83.62228263375395443, -278.3204874543079654, -213.4418079053755548 ) ) ;
#6009=CARTESIAN_POINT ( 'NONE',  ( -39.96648372379942060, -276.7509731606716059, -347.3082744206993766 ) ) ;
#6010=CARTESIAN_POINT ( 'NONE',  ( -51.60601112674886792, -279.2352042535546275, -343.8223857041643328 ) ) ;
#6011=CARTESIAN_POINT ( 'NONE',  ( 169.3709080288175528, 229.8928499549132880, -190.9150157918655282 ) ) ;
#6012=CARTESIAN_POINT ( 'NONE',  ( -17.13024629461648374, -278.8828484576725373, -196.6718825045445271 ) ) ;
#6013=CARTESIAN_POINT ( 'NONE',  ( -46.91130203267351106, -283.9502742395509927, -196.2803571052962184 ) ) ;
#6014=CARTESIAN_POINT ( 'NONE',  ( -110.6089248337608950, -298.0565533206940927, -290.5077752547692285 ) ) ;
#6015=CARTESIAN_POINT ( 'NONE',  ( 3.856251671994097574, -294.9729584840727057, -330.6994740175380798 ) ) ;
#6017=CARTESIAN_POINT ( 'NONE',  ( -60.39789375266617100, -290.4317752692833778, -200.5248081682064765 ) ) ;
#6018=CARTESIAN_POINT ( 'NONE',  ( -21.38404973707247692, -274.9030555115559196, -195.1370116052208630 ) ) ;
#6019=CARTESIAN_POINT ( 'NONE',  ( -109.8857675254993609, -272.6596122241019771, -262.2150584787953562 ) ) ;
#6025=CARTESIAN_POINT ( 'NONE',  ( 34.05833804426701050, -282.4134863947147664, -253.7400282558174354 ) ) ;
#6026=CARTESIAN_POINT ( 'NONE',  ( -90.36730959580737021, -281.0746793626499311, -215.8611060414256144 ) ) ;
#6027=CARTESIAN_POINT ( 'NONE',  ( -40.25568207211312455, -282.1484228624309480, -343.5384174535101920 ) ) ;
#6028=CARTESIAN_POINT ( 'NONE',  ( 30.08483914091539191, -282.9990922065770178, -239.1811731680289768 ) ) ;
#6029=CARTESIAN_POINT ( 'NONE',  ( 10.09572021311817736, -274.8639928247811213, -326.7561434895976618 ) ) ;
#6034=CARTESIAN_POINT ( 'NONE',  ( -108.5030311645493555, -278.9860634965922372, -299.3477318790779123 ) ) ;
#6038=CARTESIAN_POINT ( 'NONE',  ( -112.6961097755201422, -286.5364693665569575, -270.0150740228486370 ) ) ;
#6039=CARTESIAN_POINT ( 'NONE',  ( 34.10971757953186057, -292.5415648980221022, -254.5774852944237523 ) ) ;
#6040=CARTESIAN_POINT ( 'NONE',  ( 24.05581056322921185, -287.5180993374442551, -316.6607774614274149 ) ) ;
#6041=CARTESIAN_POINT ( 'NONE',  ( -106.5039957381839599, -283.1390750320503571, -244.0067847931236713 ) ) ;
#6042=CARTESIAN_POINT ( 'NONE',  ( -70.22960506001793135, -284.1847746285217795, -204.5157583719768013 ) ) ;
#6043=CARTESIAN_POINT ( 'NONE',  ( -31.81779088451380844, -287.2214873955384178, -344.2193569050722886 ) ) ;
#6044=CARTESIAN_POINT ( 'NONE',  ( -1.042353637751539219, -283.7638682205783311, -334.1536563359283036 ) ) ;
#6045=CARTESIAN_POINT ( 'NONE',  ( -2.215051817335441431, -272.5169823324737308, -204.0955973121915292 ) ) ;
#6046=CARTESIAN_POINT ( 'NONE',  ( -57.52422196158602929, -284.1958601810950427, -196.8277348213053983 ) ) ;
#6047=CARTESIAN_POINT ( 'NONE',  ( -98.31096105726601309, -299.1465021697725888, -226.6833218814015538 ) ) ;
#6048=CARTESIAN_POINT ( 'NONE',  ( -57.24536142066678224, -283.7958924575103765, -197.8234864103609141 ) ) ;
#6049=CARTESIAN_POINT ( 'NONE',  ( 0.5113351721018359886, -281.5109392116309550, -207.6082718563130811 ) ) ;
#6050=CARTESIAN_POINT ( 'NONE',  ( 20.65888604817430263, -288.8942117181810545, -222.5493994004961564 ) ) ;
#6053=CARTESIAN_POINT ( 'NONE',  ( 12.31342757672488197, -294.6573769579096620, -213.4077819255724933 ) ) ;
#6054=CARTESIAN_POINT ( 'NONE',  ( -62.48363449053908170, -275.3789563292572211, -341.0766793583003960 ) ) ;
#6055=CARTESIAN_POINT ( 'NONE',  ( -98.21405665386636485, -290.3765817901110040, -223.4493740493912242 ) ) ;
#6056=CARTESIAN_POINT ( 'NONE',  ( 10.79812279102936401, -292.7731343243028732, -326.2985639600900072 ) ) ;
#6057=CARTESIAN_POINT ( 'NONE',  ( -95.99527464800895871, -277.8551197509483472, -226.0570361621963684 ) ) ;
#6058=CARTESIAN_POINT ( 'NONE',  ( -69.77618293275435235, -295.7600024742189930, -203.5863487265986294 ) ) ;
#6059=CARTESIAN_POINT ( 'NONE',  ( -84.15596269872959567, -292.7077342042797454, -213.7071834629577722 ) ) ;
#6060=CARTESIAN_POINT ( 'NONE',  ( -106.6662871844225293, -287.4805209788416391, -237.0123917617630696 ) ) ;
#6061=CARTESIAN_POINT ( 'NONE',  ( -96.79387123168692142, -295.6789657453386440, -222.5265373234953188 ) ) ;
#6062=CARTESIAN_POINT ( 'NONE',  ( -91.16237061436491729, -291.4327915439585581, -320.9310281449119771 ) ) ;
#6063=CARTESIAN_POINT ( 'NONE',  ( -39.16461470641952047, -290.2694682189896298, -194.3834529505225532 ) ) ;
#6064=CARTESIAN_POINT ( 'NONE',  ( -84.21822483988832175, -292.8178147669369196, -213.6339961942476577 ) ) ;
#6066=CARTESIAN_POINT ( 'NONE',  ( -110.4075655545769195, -291.4158735341030706, -265.7355749416362301 ) ) ;
#6068=CARTESIAN_POINT ( 'NONE',  ( -100.3452413808355033, -291.1787881130031792, -313.9336151381815512 ) ) ;
#6069=CARTESIAN_POINT ( 'NONE',  ( 36.80257838763506584, -279.7451208784507344, -283.8875015688768144 ) ) ;
#6070=CARTESIAN_POINT ( 'NONE',  ( 35.70798575139937014, -293.5574130684050260, -270.7599229830289005 ) ) ;
#6071=CARTESIAN_POINT ( 'NONE',  ( -7.536989558263370803, -280.4322196772617417, -199.3490738489731200 ) ) ;
#6072=CARTESIAN_POINT ( 'NONE',  ( -0.3893175335183487462, -282.2414310786630836, -337.9057920514401872 ) ) ;
#6073=CARTESIAN_POINT ( 'NONE',  ( -12.70781070355129039, -286.7309927970715080, -341.0236958950612802 ) ) ;
#6074=CARTESIAN_POINT ( 'NONE',  ( 36.92364100776275393, -279.6685868693510315, -268.5771397648979359 ) ) ;
#6075=CARTESIAN_POINT ( 'NONE',  ( -31.02620414692890449, -284.1317716819260681, -195.6145403548395052 ) ) ;
#6077=CARTESIAN_POINT ( 'NONE',  ( -53.59375983348104455, -278.3273073072952002, -195.7511693299308320 ) ) ;
#6078=CARTESIAN_POINT ( 'NONE',  ( -70.91844213813423892, -284.5398077948256628, -201.4111730416956902 ) ) ;
#6079=CARTESIAN_POINT ( 'NONE',  ( 35.76383957032597749, -276.4069825415440960, -274.3111788450280528 ) ) ;
#6081=CARTESIAN_POINT ( 'NONE',  ( 7.142413368725160971, -294.2698835450690922, -211.4747523324210192 ) ) ;
#6082=CARTESIAN_POINT ( 'NONE',  ( -4.098985192281886292, -275.9071668662159595, -201.5460815532364904 ) ) ;
#6083=CARTESIAN_POINT ( 'NONE',  ( -109.0648539953097753, -278.0372349821024613, -284.1340162663009323 ) ) ;
#6084=CARTESIAN_POINT ( 'NONE',  ( -109.4745867473442615, -291.0612731992603699, -243.2676167652135177 ) ) ;
#6085=CARTESIAN_POINT ( 'NONE',  ( -87.38645428948795768, -281.8231106743042460, -327.0422776791623392 ) ) ;
#6087=CARTESIAN_POINT ( 'NONE',  ( -41.59455453792438817, -291.0561612959225499, -197.1994036284999368 ) ) ;
#6088=CARTESIAN_POINT ( 'NONE',  ( 29.11800313306291699, -292.0124013372352465, -305.1189730405533851 ) ) ;
#6091=CARTESIAN_POINT ( 'NONE',  ( -34.84890870758367498, -291.5919605982918483, -197.3421174912564027 ) ) ;
#6094=CARTESIAN_POINT ( 'NONE',  ( -105.5937364680635966, -299.2662352645559167, -254.8156830097664738 ) ) ;
#6095=CARTESIAN_POINT ( 'NONE',  ( -110.5849994635594697, -295.9025738146879689, -247.2015414032112233 ) ) ;
#6096=CARTESIAN_POINT ( 'NONE',  ( -111.0120537506639380, -285.6070266184644311, -291.0003347949233330 ) ) ;
#6097=CARTESIAN_POINT ( 'NONE',  ( 33.38909083593797789, -287.1464931707760115, -252.2508900825876026 ) ) ;
#6098=CARTESIAN_POINT ( 'NONE',  ( 36.39287900440442058, -277.0881741381935512, -271.5772722800994643 ) ) ;
#6099=CARTESIAN_POINT ( 'NONE',  ( -109.9037581196022870, -294.3456727388120839, -287.9249344330636973 ) ) ;
#6100=CARTESIAN_POINT ( 'NONE',  ( -76.17085491830529520, -297.3385052082472839, -333.4309437484569685 ) ) ;
#6102=CARTESIAN_POINT ( 'NONE',  ( 20.32495631621481991, -274.9843479026411615, -315.7871597573177951 ) ) ;
#6105=CARTESIAN_POINT ( 'NONE',  ( -108.8673779565948792, -296.5815716677780074, -241.7605266901245500 ) ) ;
#6106=CARTESIAN_POINT ( 'NONE',  ( 34.77770760792697757, -289.2329897729304662, -251.8677942383068000 ) ) ;
#6107=CARTESIAN_POINT ( 'NONE',  ( -52.18709021055299502, -295.8620628868436029, -196.7927256169245993 ) ) ;
#6108=CARTESIAN_POINT ( 'NONE',  ( 17.90801334263261069, -288.8854616061919955, -318.3050898869007597 ) ) ;
#6110=CARTESIAN_POINT ( 'NONE',  ( -82.09194440340202448, -278.5169816781325380, -207.9893627591955010 ) ) ;
#6111=CARTESIAN_POINT ( 'NONE',  ( -99.01566137253699651, -297.8155031830853545, -224.4083719213211054 ) ) ;
#6112=CARTESIAN_POINT ( 'NONE',  ( -106.1288864628091204, -289.1060797715368835, -238.4772942746835724 ) ) ;
#6113=CARTESIAN_POINT ( 'NONE',  ( -114.2887788053904217, -296.9307258127167870, -266.7405081365514548 ) ) ;
#6114=CARTESIAN_POINT ( 'NONE',  ( 34.73412790656426097, -293.7299528060083276, -258.5713172227330574 ) ) ;
#6118=CARTESIAN_POINT ( 'NONE',  ( 34.42704087534821866, -289.4043550773267270, -296.4370661045614384 ) ) ;
#6119=CARTESIAN_POINT ( 'NONE',  ( -111.2869819898779866, -275.4805209788415823, -234.7871824221999191 ) ) ;
#6121=CARTESIAN_POINT ( 'NONE',  ( 39.08244059342509047, -280.7881470642360000, -261.3701320586211523 ) ) ;
#6122=CARTESIAN_POINT ( 'NONE',  ( 13.17253473191948743, -284.3442213114847164, -325.5728966228734294 ) ) ;
#6123=CARTESIAN_POINT ( 'NONE',  ( -7.555937486864927166, -285.0096507889122677, -199.9385999065484327 ) ) ;
#6124=CARTESIAN_POINT ( 'NONE',  ( -107.3958357662211540, -288.3032179906163037, -295.5351577177019067 ) ) ;
#6125=CARTESIAN_POINT ( 'NONE',  ( 36.04826454221141319, -277.6519314244757197, -289.1818132139968043 ) ) ;
#6127=CARTESIAN_POINT ( 'NONE',  ( -103.1310101955112373, -278.1227559085914436, -302.1129792847488034 ) ) ;
#6128=CARTESIAN_POINT ( 'NONE',  ( 34.43590914722005891, -280.7173963942254886, -256.4435106977344958 ) ) ;
#6129=CARTESIAN_POINT ( 'NONE',  ( -34.28957869236049305, -278.0942853629294973, -346.9912495575085245 ) ) ;
#6130=CARTESIAN_POINT ( 'NONE',  ( -40.97413401564302404, -278.8023573981167260, -193.8312331652753642 ) ) ;
#6131=CARTESIAN_POINT ( 'NONE',  ( 159.2118730347355040, 219.5970318917149768, -203.3186411165585810 ) ) ;
#6132=CARTESIAN_POINT ( 'NONE',  ( -111.5937896373990412, -273.7403149086202916, -250.6781500681430259 ) ) ;
#6133=CARTESIAN_POINT ( 'NONE',  ( -113.6483667957982107, -274.0720294864290167, -270.3804296936822880 ) ) ;
#6134=CARTESIAN_POINT ( 'NONE',  ( -110.4542110544635705, -292.8376638359844719, -287.0812184334320705 ) ) ;
#6135=DIRECTION ( 'NONE',  ( -1.000000000000000000, -0.000000000000000000, -0.000000000000000000 ) ) ;
#6136=CARTESIAN_POINT ( 'NONE',  ( 20.61025189801298652, -289.2616779655754726, -315.2790799315228583 ) ) ;
#6137=CARTESIAN_POINT ( 'NONE',  ( -93.19039151972846469, -287.0238133388053257, -218.7582787028780729 ) ) ;
#6138=CARTESIAN_POINT ( 'NONE',  ( 35.37663929389177753, -286.8022121870467913, -262.8820953351711864 ) ) ;
#6139=CARTESIAN_POINT ( 'NONE',  ( -74.25197882986223874, -283.0365817738089618, -337.9272917728421817 ) ) ;
#6140=CARTESIAN_POINT ( 'NONE',  ( -32.89466816449868958, -278.5089819398108375, -196.6952213770649394 ) ) ;
#6141=CARTESIAN_POINT ( 'NONE',  ( 13.97661457833849141, -288.6414862554391334, -216.6497881114142103 ) ) ;
#6142=CARTESIAN_POINT ( 'NONE',  ( 34.74745710294403978, -279.8314344876043265, -255.0083958591818885 ) ) ;
#6144=CARTESIAN_POINT ( 'NONE',  ( -8.530013592997137906, -277.9821581966813824, -337.9848874139491954 ) ) ;
#6145=CARTESIAN_POINT ( 'NONE',  ( 22.32747080595033751, -275.4562334121121125, -228.1781247950915485 ) ) ;
#6146=CARTESIAN_POINT ( 'NONE',  ( 34.69380407767113894, -286.6795964428744128, -296.5709700656075256 ) ) ;
#6147=CARTESIAN_POINT ( 'NONE',  ( 6.840533778072469318, -283.2709493226794280, -333.2918303956634531 ) ) ;
#6148=CARTESIAN_POINT ( 'NONE',  ( -94.34933860692810015, -284.3418476194091795, -322.0493705473210753 ) ) ;
#6149=CARTESIAN_POINT ( 'NONE',  ( 3.391980919436260233, -282.6546167578878794, -331.0008682391191996 ) ) ;
#6153=CARTESIAN_POINT ( 'NONE',  ( -75.02837810709432631, -291.4090589529651538, -336.0879753833191330 ) ) ;
#6154=CARTESIAN_POINT ( 'NONE',  ( -50.46519167494317770, -290.5727599478697130, -194.9882300109461255 ) ) ;
#6155=CARTESIAN_POINT ( 'NONE',  ( -40.51476382051683345, -297.2084334667812868, -197.2559056900744281 ) ) ;
#6156=CARTESIAN_POINT ( 'NONE',  ( -4.553535239038832394, -293.9800174437330043, -339.9330909725131846 ) ) ;
#6159=CARTESIAN_POINT ( 'NONE',  ( -37.28675259310060852, -287.5313286789786389, -344.0544333888452115 ) ) ;
#6160=CARTESIAN_POINT ( 'NONE',  ( -9.323374709152744799, -290.6632045607491364, -201.8014872502685364 ) ) ;
#6161=CARTESIAN_POINT ( 'NONE',  ( 3.850075219107168767, -289.6892835545980347, -331.1708110788648582 ) ) ;
#6163=CARTESIAN_POINT ( 'NONE',  ( -102.8751189456563679, -293.0377465666505259, -233.8868576847403347 ) ) ;
#6164=CARTESIAN_POINT ( 'NONE',  ( -100.1379850857831570, -289.1094240273696414, -228.9560795584055199 ) ) ;
#6166=CARTESIAN_POINT ( 'NONE',  ( -56.43403404432657311, -293.8064119183956677, -197.7789372747151049 ) ) ;
#6167=CARTESIAN_POINT ( 'NONE',  ( -44.05784911650182778, -286.9064072226856865, -197.4344302004051315 ) ) ;
#6168=CARTESIAN_POINT ( 'NONE',  ( -19.83899551537457384, -294.2766665352193058, -197.2071013247608278 ) ) ;
#6172=CARTESIAN_POINT ( 'NONE',  ( -38.36100491794313427, -276.0193209134464496, -195.0128079504726770 ) ) ;
#6173=CARTESIAN_POINT ( 'NONE',  ( -114.1478250495710682, -295.7947949219372390, -266.7326872174685946 ) ) ;
#6174=CARTESIAN_POINT ( 'NONE',  ( 35.84702391920586706, -273.6475459290978733, -259.2582025667841776 ) ) ;
#6175=CARTESIAN_POINT ( 'NONE',  ( -111.5933069882814266, -276.7004617299519396, -265.0683800930034977 ) ) ;
#6176=CARTESIAN_POINT ( 'NONE',  ( -37.16513218877542357, -299.3695919249173585, -196.8650551490323721 ) ) ;
#6177=CARTESIAN_POINT ( 'NONE',  ( 9.166183792013789855, -273.2516035846269915, -209.7342013153218261 ) ) ;
#6178=CARTESIAN_POINT ( 'NONE',  ( -109.9412787060566501, -297.8200282176399014, -282.3892561632160891 ) ) ;
#6180=CARTESIAN_POINT ( 'NONE',  ( -86.21573634893285032, -298.1559647525178320, -215.9191276624551392 ) ) ;
#6182=CARTESIAN_POINT ( 'NONE',  ( -10.55455361439076434, -284.4198379758917667, -199.8721810464378450 ) ) ;
#6183=CARTESIAN_POINT ( 'NONE',  ( 8.928578900605470992, -298.6472714677322529, -197.3611204045932084 ) ) ;
#6184=CARTESIAN_POINT ( 'NONE',  ( -54.96460918990257483, -285.8315914952464141, -195.4049102596583225 ) ) ;
#6185=CARTESIAN_POINT ( 'NONE',  ( -108.7804172452479889, -289.8548615205696137, -299.0360894403287375 ) ) ;
#6186=CARTESIAN_POINT ( 'NONE',  ( -95.23130678774714397, -297.8687555266120057, -318.6222370427543638 ) ) ;
#6187=CARTESIAN_POINT ( 'NONE',  ( -39.77350657260084432, -293.0825783079234270, -345.1676751913112184 ) ) ;
#6188=CARTESIAN_POINT ( 'NONE',  ( -19.78316589113467572, -279.4693761617219252, -195.5010015131282728 ) ) ;
#6189=CARTESIAN_POINT ( 'NONE',  ( -85.33152481854862970, -287.1952119285919025, -330.4860931364851808 ) ) ;
#6191=CARTESIAN_POINT ( 'NONE',  ( -74.93237634285625859, -288.3597150576446211, -333.4161239805175114 ) ) ;
#6193=CARTESIAN_POINT ( 'NONE',  ( -90.08517449047870684, -287.7974552631008009, -323.6820947145538980 ) ) ;
#6194=CARTESIAN_POINT ( 'NONE',  ( -69.62569380259114382, -299.2199864273650292, -203.9970903007093170 ) ) ;
#6195=CARTESIAN_POINT ( 'NONE',  ( -69.72926855144149272, -281.0593605385857359, -201.1395278911332696 ) ) ;
#6196=CARTESIAN_POINT ( 'NONE',  ( -95.26367600118032897, -293.9096116816541553, -318.5833846459750021 ) ) ;
#6197=CARTESIAN_POINT ( 'NONE',  ( -8.494241580696364480, -282.6637061493995020, -337.4194816321220287 ) ) ;
#6198=CARTESIAN_POINT ( 'NONE',  ( -101.6270970665464972, -296.1604316727464266, -312.8413572493814740 ) ) ;
#6199=CARTESIAN_POINT ( 'NONE',  ( -47.38622948753410213, -299.4424650463605531, -197.3038362871796210 ) ) ;
#6200=CARTESIAN_POINT ( 'NONE',  ( 38.26126521051239138, -285.6471918085137531, -271.5534346435341604 ) ) ;
#6201=CARTESIAN_POINT ( 'NONE',  ( 21.29529204304514423, -282.9092808645379478, -223.5785050336387485 ) ) ;
#6202=CARTESIAN_POINT ( 'NONE',  ( -98.93767660563467814, -295.0633222878150832, -310.0689894473713935 ) ) ;
#6205=CARTESIAN_POINT ( 'NONE',  ( 1.988922335289990295, -284.5032803419713332, -333.8639702252353345 ) ) ;
#6207=CARTESIAN_POINT ( 'NONE',  ( -114.2704648735229114, -294.0523547857347353, -270.3284710469133074 ) ) ;
#6208=CARTESIAN_POINT ( 'NONE',  ( 20.69156538813412638, -275.4315121769824373, -320.7427095709945206 ) ) ;
#6209=CARTESIAN_POINT ( 'NONE',  ( 33.64826364582375362, -293.1603887243161921, -253.2952121250226583 ) ) ;
#6210=CARTESIAN_POINT ( 'NONE',  ( 27.05541097175026977, -282.5869969911775570, -234.5320818124958748 ) ) ;
#6211=CARTESIAN_POINT ( 'NONE',  ( 23.70272951159275721, -276.5814809697065471, -228.8653593763626475 ) ) ;
#6212=CARTESIAN_POINT ( 'NONE',  ( -44.34697730798828985, -284.5642481091381910, -346.5030432885454843 ) ) ;
#6213=CARTESIAN_POINT ( 'NONE',  ( 34.15062801828890571, -280.1291092432218193, -253.7485467657982667 ) ) ;
#6214=CARTESIAN_POINT ( 'NONE',  ( -97.68747563109087650, -279.9444796993178102, -314.9178802858327231 ) ) ;
#6215=CARTESIAN_POINT ( 'NONE',  ( -29.05963080537725673, -298.1531627655757006, -193.3611175197906675 ) ) ;
#6216=CARTESIAN_POINT ( 'NONE',  ( -1.469611089725223030, -276.4231416782081965, -338.4947604255356737 ) ) ;
#6217=CARTESIAN_POINT ( 'NONE',  ( 34.84841348972083352, -295.7073786055452729, -288.5243141987052695 ) ) ;
#6220=CARTESIAN_POINT ( 'NONE',  ( -70.29244374219243241, -293.6212690641950758, -338.5996887388874939 ) ) ;
#6221=CARTESIAN_POINT ( 'NONE',  ( 32.12227694818199097, -274.7576483826667300, -247.5544670511909828 ) ) ;
#6222=CARTESIAN_POINT ( 'NONE',  ( 1.433940854225105976, -296.0639419691735270, -336.0814148394127301 ) ) ;
#6223=CARTESIAN_POINT ( 'NONE',  ( 38.82956646151796321, -294.6490386022434222, -261.7552039642083628 ) ) ;
#6224=CARTESIAN_POINT ( 'NONE',  ( 28.65913949725213783, -290.0225726966471598, -305.7406909415886958 ) ) ;
#6225=CARTESIAN_POINT ( 'NONE',  ( -62.42781681643405989, -275.3789563287456303, -340.9195147435644913 ) ) ;
#6226=CARTESIAN_POINT ( 'NONE',  ( -101.8181059383946661, -279.9708147026288998, -307.6681781409585597 ) ) ;
#6227=CARTESIAN_POINT ( 'NONE',  ( -94.19777017212925330, -293.9621944795661079, -318.4298221417039940 ) ) ;
#6228=CARTESIAN_POINT ( 'NONE',  ( 30.89847546074621931, -282.9819856178899045, -237.3226623909828277 ) ) ;
#6229=CARTESIAN_POINT ( 'NONE',  ( -101.2541012418021467, -283.9629919314676272, -234.3484708155934300 ) ) ;
#6230=CARTESIAN_POINT ( 'NONE',  ( 162.9801456899701293, 218.5183769072534119, -204.3598628306621094 ) ) ;
#6232=CARTESIAN_POINT ( 'NONE',  ( -105.5831853876918700, -284.5657052422345146, -244.3767539095219092 ) ) ;
#6234=CARTESIAN_POINT ( 'NONE',  ( 39.22152015582132378, -282.6979308047666564, -275.6259240221770597 ) ) ;
#6235=CARTESIAN_POINT ( 'NONE',  ( -105.0737947278021949, -283.8127741602531273, -234.4652986057015482 ) ) ;
#6236=CARTESIAN_POINT ( 'NONE',  ( -104.5932386789552595, -279.9742764360261162, -233.3469210455023415 ) ) ;
#6238=CARTESIAN_POINT ( 'NONE',  ( -111.8035546382335355, -279.8617966131459980, -287.0386471357826963 ) ) ;
#6239=CARTESIAN_POINT ( 'NONE',  ( -102.0172624299486870, -298.6233781216987495, -301.5434626090942061 ) ) ;
#6240=CARTESIAN_POINT ( 'NONE',  ( 6.552877139890185276, -58.82689968973230066, -354.7915936803940440 ) ) ;
#6241=CARTESIAN_POINT ( 'NONE',  ( -43.66173072863657723, -275.9724079497053708, -195.7431512892062244 ) ) ;
#6242=CARTESIAN_POINT ( 'NONE',  ( -40.04897441879919739, -139.4172891678365147, -364.6093070308725146 ) ) ;
#6243=CARTESIAN_POINT ( 'NONE',  ( -86.54999248270378587, -277.3845387750056943, -214.2327760912575059 ) ) ;
#6244=CARTESIAN_POINT ( 'NONE',  ( -47.62869337901483391, -293.6833694503192760, -195.0209006136624055 ) ) ;
#6245=CARTESIAN_POINT ( 'NONE',  ( 20.26834423938420215, -292.2671166490576411, -225.3411227970795494 ) ) ;
#6246=CARTESIAN_POINT ( 'NONE',  ( -107.6776610608314968, -289.6600801961170646, -301.6751773711759483 ) ) ;
#6248=CARTESIAN_POINT ( 'NONE',  ( 31.68984879413996936, -292.5513641340801883, -303.2449169963102804 ) ) ;
#6249=CARTESIAN_POINT ( 'NONE',  ( -88.23158215116959013, -283.7248238893824919, -216.9133834972275281 ) ) ;
#6250=CARTESIAN_POINT ( 'NONE',  ( -25.23052456769790197, -294.0684639767140425, -197.0681748386716663 ) ) ;
#6251=CARTESIAN_POINT ( 'NONE',  ( 17.41867432603079280, -285.3323989892099348, -221.0268684639362959 ) ) ;
#6252=CARTESIAN_POINT ( 'NONE',  ( -48.38637779903434222, -284.5108580119427302, -343.0196245194444487 ) ) ;
#6254=CARTESIAN_POINT ( 'NONE',  ( -104.4102421220612626, -291.9790085570930387, -233.0163608248011542 ) ) ;
#6255=CARTESIAN_POINT ( 'NONE',  ( 21.06287138854959551, -282.6605938335546284, -314.2782001541225441 ) ) ;
#6256=CARTESIAN_POINT ( 'NONE',  ( 21.96940025529735863, -293.0014218570613593, -318.8605875491716120 ) ) ;
#6257=CARTESIAN_POINT ( 'NONE',  ( 7.847822175835530878, -289.2554568675022324, -332.5722591529842020 ) ) ;
#6258=CARTESIAN_POINT ( 'NONE',  ( -41.75075935475646816, -289.5986145386717681, -347.1863540663700292 ) ) ;
#6259=CARTESIAN_POINT ( 'NONE',  ( 34.75955622041164617, -287.8705284256029699, -281.8604621962559804 ) ) ;
#6261=CARTESIAN_POINT ( 'NONE',  ( -53.01028712946499155, -297.1112087489473197, -344.5417064347121254 ) ) ;
#6262=CARTESIAN_POINT ( 'NONE',  ( -103.4154014400012613, -295.7432781014155694, -231.6877970420247266 ) ) ;
#6264=CARTESIAN_POINT ( 'NONE',  ( -97.84996783214617722, -277.0387620476395796, -311.6183353842870360 ) ) ;
#6265=CARTESIAN_POINT ( 'NONE',  ( -83.53813120887681976, -272.9455414199836696, -208.7687025647727808 ) ) ;
#6266=CARTESIAN_POINT ( 'NONE',  ( -92.72440893625083902, -294.3446140339749491, -318.9765817632398921 ) ) ;
#6267=CARTESIAN_POINT ( 'NONE',  ( 36.59802255558142292, -277.2563129351966040, -266.0580193050591333 ) ) ;
#6268=CARTESIAN_POINT ( 'NONE',  ( -68.78455360860226619, -271.7739958817561501, -203.0997926502641349 ) ) ;
#6269=CARTESIAN_POINT ( 'NONE',  ( -82.59261759771673894, -296.8910101619217130, -328.2141840206216443 ) ) ;
#6270=CARTESIAN_POINT ( 'NONE',  ( -58.48430324165660465, -296.4117015425314321, -340.5552516868115731 ) ) ;
#6272=CARTESIAN_POINT ( 'NONE',  ( -41.87735862997656255, -296.7083938070172735, -346.4778624229456341 ) ) ;
#6273=CARTESIAN_POINT ( 'NONE',  ( -110.1981243275524776, -294.3143545430784229, -288.9055788577369412 ) ) ;
#6274=CARTESIAN_POINT ( 'NONE',  ( -34.77200720577003068, -298.7349428432619902, -193.4627744701153063 ) ) ;
#6275=CARTESIAN_POINT ( 'NONE',  ( -110.7116589345665574, -289.0444136629508307, -276.6624422077042027 ) ) ;
#6276=CARTESIAN_POINT ( 'NONE',  ( -90.68200146038972775, -275.2960776682443793, -217.6371869676937365 ) ) ;
#6277=CARTESIAN_POINT ( 'NONE',  ( -96.89243378546807151, -273.6992627285809476, -221.6246768237465972 ) ) ;
#6278=CARTESIAN_POINT ( 'NONE',  ( -109.7577688912325442, -297.0141879662068618, -260.5981190934437564 ) ) ;
#6279=CARTESIAN_POINT ( 'NONE',  ( -56.17057519999156767, -281.7908150504746914, -197.3423624808561954 ) ) ;
#6280=CARTESIAN_POINT ( 'NONE',  ( -1.352514652375625293, -279.2041695886023831, -202.8475874680449920 ) ) ;
#6282=CARTESIAN_POINT ( 'NONE',  ( -13.46147542462112234, -282.0985928901151851, -343.4572714688465567 ) ) ;
#6283=CARTESIAN_POINT ( 'NONE',  ( 32.92326280345081102, -275.3000388853212712, -301.6044816060531844 ) ) ;
#6284=CARTESIAN_POINT ( 'NONE',  ( 33.83292856169706653, -280.3001911706344913, -297.5753173070963271 ) ) ;
#6285=CARTESIAN_POINT ( 'NONE',  ( -4.436608332239877051, -278.4845707366590091, -202.7652633982403358 ) ) ;
#6286=CARTESIAN_POINT ( 'NONE',  ( -16.45619101152840713, -272.9019854118938042, -199.7447425639570611 ) ) ;
#6287=CARTESIAN_POINT ( 'NONE',  ( 15.88758394768271742, -276.8059586878206915, -217.4524412971409504 ) ) ;
#6290=CARTESIAN_POINT ( 'NONE',  ( -101.4492966493872643, -295.3338736476267741, -229.5666320672262088 ) ) ;
#6291=CARTESIAN_POINT ( 'NONE',  ( -28.02685870437271731, -290.1898058533752192, -195.5313156700128161 ) ) ;
#6293=CARTESIAN_POINT ( 'NONE',  ( -39.21169192941987092, -292.0293247714836866, -193.3707930653487779 ) ) ;
#6294=CARTESIAN_POINT ( 'NONE',  ( 4.863448004814641124, -278.4835506810384800, -332.5604258201134371 ) ) ;
#6295=CARTESIAN_POINT ( 'NONE',  ( 12.90482552054991494, -272.7529408077393214, -214.6109427262394433 ) ) ;
#6297=CARTESIAN_POINT ( 'NONE',  ( -41.46562291945573975, -285.0237180993015045, -345.8598487995611208 ) ) ;
#6300=CARTESIAN_POINT ( 'NONE',  ( -30.47579335792610067, -284.1386902370635994, -195.6246995904763537 ) ) ;
#6302=CARTESIAN_POINT ( 'NONE',  ( 24.75504968184727517, -292.8858231087979789, -309.5861391591930101 ) ) ;
#6303=CARTESIAN_POINT ( 'NONE',  ( 7.694784159547886304, -284.8135216979944744, -211.2827605389728660 ) ) ;
#6305=CARTESIAN_POINT ( 'NONE',  ( -81.34832271378733992, -293.6504158052019307, -331.0934636854557311 ) ) ;
#6306=CARTESIAN_POINT ( 'NONE',  ( -113.6620627366040566, -283.0011575231761753, -272.8075153160856416 ) ) ;
#6307=CARTESIAN_POINT ( 'NONE',  ( -94.57370232682005451, -280.8046222277030779, -223.7677886117756998 ) ) ;
#6308=CARTESIAN_POINT ( 'NONE',  ( -68.35414295259512585, -286.8588275941886536, -200.3022776908047149 ) ) ;
#6309=CARTESIAN_POINT ( 'NONE',  ( 18.43182106296206868, -279.0797130265393093, -218.7540608304223611 ) ) ;
#6310=CARTESIAN_POINT ( 'NONE',  ( 23.53406431666785181, -286.9920877096481036, -229.9813714228226615 ) ) ;
#6311=CARTESIAN_POINT ( 'NONE',  ( -64.53412166755546764, -278.8393573761998709, -338.7961243743629893 ) ) ;
#6312=CARTESIAN_POINT ( 'NONE',  ( -105.6687549706312268, -279.7051851485769021, -244.0654836626166002 ) ) ;
#6313=CARTESIAN_POINT ( 'NONE',  ( -92.72830435243361080, -287.2435288401311482, -219.1893038560930336 ) ) ;
#6315=CARTESIAN_POINT ( 'NONE',  ( -100.7494579649421809, -296.9624811853774986, -226.6520661668976970 ) ) ;
#6316=CARTESIAN_POINT ( 'NONE',  ( -61.77001590052017832, -291.3510959274530592, -340.8955364608238483 ) ) ;
#6317=LINE ( 'NONE', #22371, #30712 ) ;
#6318=CARTESIAN_POINT ( 'NONE',  ( -99.90806341382572953, -281.6948066931272479, -220.5068182859052968 ) ) ;
#6320=CARTESIAN_POINT ( 'NONE',  ( 16.78750067991459005, -272.8198321972170106, -218.1321975868983714 ) ) ;
#6321=CARTESIAN_POINT ( 'NONE',  ( 28.86934481696277999, -292.4482019360023628, -308.1842068824824423 ) ) ;
#6322=CARTESIAN_POINT ( 'NONE',  ( -68.06769175122421700, -297.1451674423810232, -204.0609288307133227 ) ) ;
#6323=CARTESIAN_POINT ( 'NONE',  ( 36.14489191360531350, -289.1527651609409872, -276.5201938796278114 ) ) ;
#6324=CARTESIAN_POINT ( 'NONE',  ( -3.909623003421586862, -282.2594526982080083, -204.3146934355341386 ) ) ;
#6325=CARTESIAN_POINT ( 'NONE',  ( -26.21231425154518391, -290.3383924064307848, -345.9570375926600718 ) ) ;
#6326=CARTESIAN_POINT ( 'NONE',  ( -59.86600736562991187, -290.6532265288823851, -343.4771480662135446 ) ) ;
#6327=CARTESIAN_POINT ( 'NONE',  ( -110.9372650422978239, -286.3668230351922830, -284.8073450568668363 ) ) ;
#6328=CARTESIAN_POINT ( 'NONE',  ( -112.4022064887643069, -278.9336063995078803, -253.1878716552984940 ) ) ;
#6330=CARTESIAN_POINT ( 'NONE',  ( -14.24588526452056314, -292.8347719327491632, -342.3048288401560058 ) ) ;
#6331=CARTESIAN_POINT ( 'NONE',  ( -1.133560081756077365, -280.3524779540862824, -202.4054662756805669 ) ) ;
#6332=CARTESIAN_POINT ( 'NONE',  ( -79.57696797711281533, -275.3356402232845994, -209.2491131851420221 ) ) ;
#6333=CARTESIAN_POINT ( 'NONE',  ( 30.89617123739170168, -283.8376638359844719, -254.7536222014695397 ) ) ;
#6334=CARTESIAN_POINT ( 'NONE',  ( 37.73002525306241495, -273.6419601848323850, -258.5208129215013741 ) ) ;
#6336=CARTESIAN_POINT ( 'NONE',  ( 35.41424597613864478, -280.9647754071460213, -263.1515018985282950 ) ) ;
#6337=CARTESIAN_POINT ( 'NONE',  ( -113.3252823047819078, -279.8845142694431161, -260.2356444982568178 ) ) ;
#6338=CARTESIAN_POINT ( 'NONE',  ( -89.60455371904160415, -274.6112016343289497, -218.6906466064376673 ) ) ;
#6339=CARTESIAN_POINT ( 'NONE',  ( -68.39455665404544504, -284.7128468580357321, -200.1432233888308474 ) ) ;
#6340=CARTESIAN_POINT ( 'NONE',  ( -98.94179838893420253, -291.7502386729644286, -311.4134617236118743 ) ) ;
#6341=CARTESIAN_POINT ( 'NONE',  ( -41.17314852266008529, -275.6049439593288639, -194.2057856069723698 ) ) ;
#6342=CARTESIAN_POINT ( 'NONE',  ( -113.8491716523808606, -273.9029761287944211, -267.5287256790753077 ) ) ;
#6344=CARTESIAN_POINT ( 'NONE',  ( -109.9600571257703621, -298.7855627628606499, -252.2364317070156972 ) ) ;
#6345=CARTESIAN_POINT ( 'NONE',  ( -109.8763797858160132, -282.3150227144888049, -288.7662443556450285 ) ) ;
#6346=CARTESIAN_POINT ( 'NONE',  ( -64.37740095122899220, -291.3756458193047365, -198.2298954611370618 ) ) ;
#6347=CARTESIAN_POINT ( 'NONE',  ( 18.53315906116852574, -272.8799483769689687, -220.7885683032928625 ) ) ;
#6348=CARTESIAN_POINT ( 'NONE',  ( 15.72728003122717944, -288.3886207526388148, -215.6790938879539681 ) ) ;
#6349=CARTESIAN_POINT ( 'NONE',  ( -106.3280840637525841, -289.1435652046810674, -295.1624265110764895 ) ) ;
#6350=ORIENTED_EDGE ( 'NONE', *, *, #86805, .T. ) ;
#6351=CARTESIAN_POINT ( 'NONE',  ( -105.4704622536337268, -289.5770984406296407, -235.6456915098612228 ) ) ;
#6352=CARTESIAN_POINT ( 'NONE',  ( -98.31485524360265060, -290.7770457921772049, -230.0901575075713481 ) ) ;
#6354=CARTESIAN_POINT ( 'NONE',  ( 37.71812022522413343, -288.4334691967059712, -254.5649487843805616 ) ) ;
#6355=CARTESIAN_POINT ( 'NONE',  ( -45.90636683028166232, -277.4968833149300735, -342.9288870741538062 ) ) ;
#6356=CARTESIAN_POINT ( 'NONE',  ( -36.29252458990619346, -293.9596585521684347, -347.0578816674728273 ) ) ;
#6357=CARTESIAN_POINT ( 'NONE',  ( -37.30596059985554547, -283.7030888800183561, -347.2722252779598762 ) ) ;
#6359=CARTESIAN_POINT ( 'NONE',  ( -49.34561905264056492, -286.2365589357607405, -194.2702331627579895 ) ) ;
#6360=CARTESIAN_POINT ( 'NONE',  ( -38.88127076147136307, -283.4052399362169012, -343.3785247585709044 ) ) ;
#6361=CARTESIAN_POINT ( 'NONE',  ( 193.9776679813659825, 279.2223312090847571, -125.8845065936893519 ) ) ;
#6363=CARTESIAN_POINT ( 'NONE',  ( 120.2832162277302928, 149.7717564229777452, -262.6457934689295257 ) ) ;
#6364=CARTESIAN_POINT ( 'NONE',  ( -70.99751101762201699, -195.4794272351117854, -356.7654148836441550 ) ) ;
#6366=CARTESIAN_POINT ( 'NONE',  ( -110.0450955006309073, -271.8569090480607429, -262.1868884703152389 ) ) ;
#6367=CARTESIAN_POINT ( 'NONE',  ( -27.23401272400323947, -273.1038180833474485, -197.7010456017354727 ) ) ;
#6368=CARTESIAN_POINT ( 'NONE',  ( -44.79590847252431018, -294.6516264851212554, -346.9909908257032498 ) ) ;
#6369=CARTESIAN_POINT ( 'NONE',  ( 185.6221890035897957, 260.3163244210543894, -151.2547347512914087 ) ) ;
#6370=CARTESIAN_POINT ( 'NONE',  ( -32.69570777663797401, -272.7943540709913464, -193.9823982106830726 ) ) ;
#6371=CARTESIAN_POINT ( 'NONE',  ( -110.3527260578513420, -298.2374949657886418, -283.8573451078446510 ) ) ;
#6372=CARTESIAN_POINT ( 'NONE',  ( -106.8687973730433214, -291.9392068475891051, -247.1187252012099975 ) ) ;
#6374=CARTESIAN_POINT ( 'NONE',  ( -101.4252126843175574, -296.9348787030529593, -312.7197856971699252 ) ) ;
#6376=CARTESIAN_POINT ( 'NONE',  ( 20.40996426792068874, -288.6744489616175429, -315.1332895037521098 ) ) ;
#6377=CARTESIAN_POINT ( 'NONE',  ( 26.38355116495089092, -294.9218142523610027, -313.2942190597748322 ) ) ;
#6378=CARTESIAN_POINT ( 'NONE',  ( -68.19574210533816938, -295.9389810308233564, -340.8420018948996812 ) ) ;
#6379=CARTESIAN_POINT ( 'NONE',  ( 20.99252186944289278, -293.1025300162912686, -226.4735508539140483 ) ) ;
#6381=CARTESIAN_POINT ( 'NONE',  ( 10.84814376549343073, -276.6323434020482068, -212.0947518564657628 ) ) ;
#6384=CARTESIAN_POINT ( 'NONE',  ( -100.1950907265145219, -278.6474338818921410, -225.9879482334482077 ) ) ;
#6385=CARTESIAN_POINT ( 'NONE',  ( 35.25216680377810974, -276.3662346058220010, -260.6895652641109109 ) ) ;
#6386=CARTESIAN_POINT ( 'NONE',  ( 8.876014119766217902, -276.4365044255048929, -210.0461372479127249 ) ) ;
#6387=CARTESIAN_POINT ( 'NONE',  ( 15.77750456023545311, -274.3251199324144523, -323.8825923905679360 ) ) ;
#6388=CARTESIAN_POINT ( 'NONE',  ( -109.3777171770042003, -297.3674176332897332, -257.9230748851302906 ) ) ;
#6389=CARTESIAN_POINT ( 'NONE',  ( -107.4360443860469587, -294.8301362287202778, -292.9350903186063420 ) ) ;
#6391=CARTESIAN_POINT ( 'NONE',  ( -111.3795896698812129, -278.7820147490118643, -291.2876039639390910 ) ) ;
#6392=CARTESIAN_POINT ( 'NONE',  ( -32.41843851904511808, -277.1551741134557574, -343.2448779112194757 ) ) ;
#6393=CARTESIAN_POINT ( 'NONE',  ( 7.270050870308891966, -285.3305706223928269, -208.1420976282661286 ) ) ;
#6394=CARTESIAN_POINT ( 'NONE',  ( -90.36086187770479228, -299.3040049418938793, -217.0788797345456658 ) ) ;
#6396=CARTESIAN_POINT ( 'NONE',  ( 10.21247993001296095, -287.5739136560483757, -326.0266720910582308 ) ) ;
#6397=CARTESIAN_POINT ( 'NONE',  ( -60.02314603951818128, -277.9941401691420424, -199.8547827550420664 ) ) ;
#6398=CARTESIAN_POINT ( 'NONE',  ( -69.98546011304092929, -278.1882153518149039, -204.3944536736410953 ) ) ;
#6399=CARTESIAN_POINT ( 'NONE',  ( -96.28254124675709136, -287.1892794189643041, -223.9621247545893823 ) ) ;
#6400=CARTESIAN_POINT ( 'NONE',  ( -45.93946161100708991, -278.3685373940209615, -343.3037808704696658 ) ) ;
#6402=CARTESIAN_POINT ( 'NONE',  ( -99.64763134665689392, -276.2093950354652065, -313.8576115120782788 ) ) ;
#6403=CARTESIAN_POINT ( 'NONE',  ( 0.6583803595884690774, -275.2248800559200390, -207.9120463234600322 ) ) ;
#6404=CARTESIAN_POINT ( 'NONE',  ( 37.06030502173798880, -283.6893232537964309, -281.0555116736185823 ) ) ;
#6406=CARTESIAN_POINT ( 'NONE',  ( -2.443645688494237245, -290.5142534318678145, -337.3793244423686701 ) ) ;
#6407=CARTESIAN_POINT ( 'NONE',  ( -39.96265140076453548, -290.0190892058981831, -195.3943436893948729 ) ) ;
#6409=CARTESIAN_POINT ( 'NONE',  ( -64.73716579658461967, -272.3716022403888815, -202.1512734879954110 ) ) ;
#6410=CARTESIAN_POINT ( 'NONE',  ( 34.85450400292089057, -291.4669269607801994, -253.0274554578853099 ) ) ;
#6411=CARTESIAN_POINT ( 'NONE',  ( 125.5584997210034572, 149.0310057319917405, -265.9501514013184078 ) ) ;
#6413=CARTESIAN_POINT ( 'NONE',  ( -34.71029200711424068, -287.4995322846278327, -346.6224020364168155 ) ) ;
#6414=CARTESIAN_POINT ( 'NONE',  ( -71.76416114868720797, -285.1152112257479985, -335.6415483885547246 ) ) ;
#6415=CARTESIAN_POINT ( 'NONE',  ( 30.52691738745054550, -285.3464304731541006, -236.1876667690419822 ) ) ;
#6416=CARTESIAN_POINT ( 'NONE',  ( -95.57164275853696722, -285.3487231044622945, -315.3777781046228483 ) ) ;
#6417=CARTESIAN_POINT ( 'NONE',  ( -78.45895826735632284, -284.4243568622601401, -330.8753544044073465 ) ) ;
#6418=CARTESIAN_POINT ( 'NONE',  ( -25.30945435920438769, -294.1847050145924527, -195.9727327191242807 ) ) ;
#6419=CARTESIAN_POINT ( 'NONE',  ( 38.26621618836384897, -273.6424438104039041, -271.1808900032881979 ) ) ;
#6421=CARTESIAN_POINT ( 'NONE',  ( -55.33279510528596035, -274.1600756565751453, -195.5141755402892443 ) ) ;
#6423=CARTESIAN_POINT ( 'NONE',  ( -106.4249218411305549, -288.2325030944798527, -301.0974593380055921 ) ) ;
#6424=CARTESIAN_POINT ( 'NONE',  ( -62.40599122933164011, -277.3692701495346000, -343.2238910260608122 ) ) ;
#6425=CARTESIAN_POINT ( 'NONE',  ( 11.38383135535448254, -296.3525786689033339, -326.9090567730179373 ) ) ;
#6427=CARTESIAN_POINT ( 'NONE',  ( -97.94846578770459189, -282.6611630872141063, -312.0198232531813005 ) ) ;
#6429=CARTESIAN_POINT ( 'NONE',  ( -96.11335332297561251, -277.1921505493837117, -223.7682705236798597 ) ) ;
#6431=CARTESIAN_POINT ( 'NONE',  ( -71.07868559826272303, -272.0948510084914460, -201.9175385404270173 ) ) ;
#6432=CARTESIAN_POINT ( 'NONE',  ( -108.8662258347256824, -277.7017663279243607, -285.4652528791221471 ) ) ;
#6434=CARTESIAN_POINT ( 'NONE',  ( -4.005868003585892900, -296.1244270264804754, -336.0976216752981145 ) ) ;
#6435=CARTESIAN_POINT ( 'NONE',  ( -1.268629040287204024, -279.4396341413352616, -202.6837506229804831 ) ) ;
#6436=CARTESIAN_POINT ( 'NONE',  ( 35.76874303303664959, -294.4267036498310404, -265.2881402944820479 ) ) ;
#6437=CARTESIAN_POINT ( 'NONE',  ( -19.38665920633425799, -296.1411593032297560, -344.7857749897622170 ) ) ;
#6438=CARTESIAN_POINT ( 'NONE',  ( -100.7340143359106577, -272.7165427928381973, -234.0171802570863804 ) ) ;
#6439=CARTESIAN_POINT ( 'NONE',  ( -96.51316919855044318, -291.9200719114670619, -316.4658879937258575 ) ) ;
#6440=CARTESIAN_POINT ( 'NONE',  ( -57.75797785678248886, -285.9623842389826223, -196.0617384996037060 ) ) ;
#6441=CARTESIAN_POINT ( 'NONE',  ( -73.33680312742842489, -271.7199786854134231, -203.6345357088191861 ) ) ;
#6442=CARTESIAN_POINT ( 'NONE',  ( 39.64009771593815401, -287.3645348205320147, -268.6869599293588067 ) ) ;
#6443=CARTESIAN_POINT ( 'NONE',  ( -108.0098986598259785, -280.8463087524490334, -246.1636644110311067 ) ) ;
#6445=CARTESIAN_POINT ( 'NONE',  ( -71.27663862723254340, -284.6512386791011409, -205.4625170904564300 ) ) ;
#6446=CARTESIAN_POINT ( 'NONE',  ( -23.70134904317697888, -286.8778148163198694, -344.1630038626366286 ) ) ;
#6447=CARTESIAN_POINT ( 'NONE',  ( 117.8046289747227320, 148.0164379187816053, -257.9426961570557069 ) ) ;
#6448=CARTESIAN_POINT ( 'NONE',  ( 16.94053583275968577, -286.3600077972337203, -221.4402168874307222 ) ) ;
#6449=CARTESIAN_POINT ( 'NONE',  ( 29.56273004993958864, -282.9844407478719859, -308.1074613971295548 ) ) ;
#6450=CARTESIAN_POINT ( 'NONE',  ( -112.3380454106139723, -289.4053982281808999, -286.7430717223928696 ) ) ;
#6451=CARTESIAN_POINT ( 'NONE',  ( -53.60976510433307851, -281.4470555692896028, -195.8639101480814020 ) ) ;
#6452=CARTESIAN_POINT ( 'NONE',  ( -94.60388262250833691, -280.5591372041472482, -219.6231565594009112 ) ) ;
#6453=CARTESIAN_POINT ( 'NONE',  ( 20.17965966133159483, -282.0190265935351590, -315.3087894741240120 ) ) ;
#6454=CARTESIAN_POINT ( 'NONE',  ( 37.58354874936826207, -277.4962935480174337, -265.9979052796920200 ) ) ;
#6455=CARTESIAN_POINT ( 'NONE',  ( -44.79562445103660906, -295.1438942955880975, -347.0528897455528750 ) ) ;
#6456=CARTESIAN_POINT ( 'NONE',  ( -10.14786510462004010, -286.7156592088262528, -339.9315967635010907 ) ) ;
#6457=CARTESIAN_POINT ( 'NONE',  ( 3.812560456761368677, -296.1086018564839719, -334.5541116968458937 ) ) ;
#6458=CARTESIAN_POINT ( 'NONE',  ( -101.7454054937444567, -294.9965075280497899, -305.3809524760209797 ) ) ;
#6461=CARTESIAN_POINT ( 'NONE',  ( 35.05627616331315011, -283.6970158355071590, -287.7315179273286390 ) ) ;
#6462=CARTESIAN_POINT ( 'NONE',  ( -109.2959700491762760, -296.3828823077925563, -257.9244573800945091 ) ) ;
#6463=CARTESIAN_POINT ( 'NONE',  ( 38.51284071453761015, -294.7736513591875109, -281.6563002893304315 ) ) ;
#6464=CARTESIAN_POINT ( 'NONE',  ( -29.42538135728312909, -283.6007878141642209, -343.0837265835177732 ) ) ;
#6465=CARTESIAN_POINT ( 'NONE',  ( -44.01033522066330050, -273.0286825488211093, -193.8334704915201883 ) ) ;
#6466=CARTESIAN_POINT ( 'NONE',  ( 10.17148705544911103, -289.0681354844280122, -330.8921587932057946 ) ) ;
#6467=CARTESIAN_POINT ( 'NONE',  ( -105.8981936611681789, -282.2718806229563029, -302.6149963885009697 ) ) ;
#6468=CARTESIAN_POINT ( 'NONE',  ( -97.27093951715011144, -290.2373663458233750, -318.6957797608142187 ) ) ;
#6469=CARTESIAN_POINT ( 'NONE',  ( 34.54325119434125213, -288.0546513150305259, -283.1923790351183925 ) ) ;
#6472=CARTESIAN_POINT ( 'NONE',  ( -82.51230583331636126, -218.8770980360667693, -348.9302519833477731 ) ) ;
#6473=CARTESIAN_POINT ( 'NONE',  ( 39.58706461736021254, -273.0523547857348490, -270.3937649182068981 ) ) ;
#6474=CARTESIAN_POINT ( 'NONE',  ( -103.5115380187420584, -278.1715385815084005, -239.0306326137186375 ) ) ;
#6475=VERTEX_POINT ( 'NONE', #15211 ) ;
#6476=CARTESIAN_POINT ( 'NONE',  ( -35.64190526219495325, -278.9942678978713957, -197.0592586586642483 ) ) ;
#6477=CARTESIAN_POINT ( 'NONE',  ( 28.48666950001588205, -274.6966934687411026, -230.3546945851999226 ) ) ;
#6478=CARTESIAN_POINT ( 'NONE',  ( -64.98731406889790208, -279.4141527825871663, -339.9556852273502159 ) ) ;
#6479=CARTESIAN_POINT ( 'NONE',  ( -29.06568833929538798, -125.6893641773768877, -361.8808603065265856 ) ) ;
#6480=CARTESIAN_POINT ( 'NONE',  ( -112.6526487677783166, -277.2896839759220597, -257.4434050069697264 ) ) ;
#6481=CARTESIAN_POINT ( 'NONE',  ( -83.83854698117650628, -281.7138610158831398, -328.8217258226717377 ) ) ;
#6482=CARTESIAN_POINT ( 'NONE',  ( -98.29321305435765055, -298.9240519474489020, -224.9644325659491813 ) ) ;
#6483=CARTESIAN_POINT ( 'NONE',  ( 30.64512757076958849, -294.4036246806608119, -297.2536289764103685 ) ) ;
#6485=CARTESIAN_POINT ( 'NONE',  ( -93.80805598178397986, -289.9001162951274750, -223.3011317145225121 ) ) ;
#6486=CARTESIAN_POINT ( 'NONE',  ( 36.48565114859932379, -275.9313006778426711, -248.6615087708247529 ) ) ;
#6487=CARTESIAN_POINT ( 'NONE',  ( -110.3417001280813849, -272.5880843968022873, -267.6372586758525927 ) ) ;
#6490=CIRCLE ( 'NONE', #36684, 1.000000000000000888 ) ;
#6493=CARTESIAN_POINT ( 'NONE',  ( 26.72232934394043014, -282.1466173397262764, -234.7236910181440237 ) ) ;
#6494=CARTESIAN_POINT ( 'NONE',  ( 18.40135289542600106, -282.5994273224870312, -218.7211523205825188 ) ) ;
#6495=CARTESIAN_POINT ( 'NONE',  ( -108.6571634405473645, -283.3911927967691327, -287.0746750277188539 ) ) ;
#6496=CARTESIAN_POINT ( 'NONE',  ( 14.17553149012710634, -282.6450427156368619, -216.8400868703600395 ) ) ;
#6497=CARTESIAN_POINT ( 'NONE',  ( 16.08735612131448889, -274.7568267279347083, -321.1158586555979468 ) ) ;
#6502=CARTESIAN_POINT ( 'NONE',  ( -89.09579538521494158, -278.5611536762490914, -327.1561216729629678 ) ) ;
#6505=ORIENTED_EDGE ( 'NONE', *, *, #60912, .F. ) ;
#6507=CARTESIAN_POINT ( 'NONE',  ( -110.7629702859770049, -286.7488097006516909, -253.3986919732841159 ) ) ;
#6508=CARTESIAN_POINT ( 'NONE',  ( 35.80294670404060042, -292.7907103614479638, -273.5060859757203389 ) ) ;
#6510=CARTESIAN_POINT ( 'NONE',  ( 19.54324741911989349, -287.6050977731702574, -322.1244776297479575 ) ) ;
#6511=CARTESIAN_POINT ( 'NONE',  ( -33.15928537565051215, -284.3452565886557295, -196.4155367775724699 ) ) ;
#6512=CARTESIAN_POINT ( 'NONE',  ( -75.00622501962587307, -284.1144807241320223, -207.1411964243589807 ) ) ;
#6513=CARTESIAN_POINT ( 'NONE',  ( -97.39374860989762794, -288.1952892120093566, -313.6245608417328867 ) ) ;
#6514=CARTESIAN_POINT ( 'NONE',  ( -33.45996125047639680, -284.2073162824495967, -343.6681147690134139 ) ) ;
#6515=CARTESIAN_POINT ( 'NONE',  ( -35.54547121304181445, -272.0745038785823340, -195.3698374586679734 ) ) ;
#6516=CARTESIAN_POINT ( 'NONE',  ( -110.3474330995260999, -282.6746769152262004, -292.2377169337230498 ) ) ;
#6517=CARTESIAN_POINT ( 'NONE',  ( -73.61611860142298269, -297.5333320825926648, -336.0635182075294551 ) ) ;
#6518=CARTESIAN_POINT ( 'NONE',  ( -40.70824095597872372, -284.0098745121070465, -195.2189231717056828 ) ) ;
#6519=CARTESIAN_POINT ( 'NONE',  ( -105.4823552742332851, -279.1356499873536450, -297.1987699638935396 ) ) ;
#6520=CARTESIAN_POINT ( 'NONE',  ( 0.5743636803178351347, -288.5564003807857034, -205.4431388171454387 ) ) ;
#6522=CARTESIAN_POINT ( 'NONE',  ( 129.8975571001389540, -299.5541904835127980, -201.2022030660758389 ) ) ;
#6523=CARTESIAN_POINT ( 'NONE',  ( 33.11769049971713486, -295.8246267347387857, -297.6519308754502049 ) ) ;
#6526=CARTESIAN_POINT ( 'NONE',  ( -67.63316614681787087, -275.4494358090855144, -338.9718149474385882 ) ) ;
#6527=CARTESIAN_POINT ( 'NONE',  ( -112.7116143465756437, -289.5611102020022827, -285.3789357411529295 ) ) ;
#6528=CARTESIAN_POINT ( 'NONE',  ( -78.41168134439851656, -294.0145096028305716, -331.7392226573571747 ) ) ;
#6529=CARTESIAN_POINT ( 'NONE',  ( -67.49339956153842479, -278.3329741898783141, -203.3241532024158573 ) ) ;
#6530=CARTESIAN_POINT ( 'NONE',  ( -47.41733740621171478, -296.0624716098051863, -196.7607795853814423 ) ) ;
#6531=CARTESIAN_POINT ( 'NONE',  ( -2.218387250261451449, -293.8424804235529564, -205.7899047976282816 ) ) ;
#6532=CARTESIAN_POINT ( 'NONE',  ( -106.6379572354042153, -280.6233781216988064, -303.7686719486574134 ) ) ;
#6533=CARTESIAN_POINT ( 'NONE',  ( -6.099435426505046109, -293.1288594594918209, -339.9788502848842313 ) ) ;
#6534=CARTESIAN_POINT ( 'NONE',  ( 8.492553830895174016, -290.0124198531250954, -328.2028120882733333 ) ) ;
#6535=CARTESIAN_POINT ( 'NONE',  ( 24.00972035802857718, -291.1888897783472885, -225.5283484969783956 ) ) ;
#6536=CARTESIAN_POINT ( 'NONE',  ( -31.80908460157409223, -290.4063869104180071, -343.7931086499631874 ) ) ;
#6538=CARTESIAN_POINT ( 'NONE',  ( -92.52680752193022329, -290.6709314837173679, -318.4701931679086897 ) ) ;
#6540=CARTESIAN_POINT ( 'NONE',  ( -110.3984837575261224, -291.4642496548331678, -293.5715511321573672 ) ) ;
#6541=CARTESIAN_POINT ( 'NONE',  ( 36.25357655829716919, -279.7799331761949588, -286.6114207950956256 ) ) ;
#6542=CARTESIAN_POINT ( 'NONE',  ( 34.32437576633277132, -293.7354040298964719, -284.2526105552130957 ) ) ;
#6543=CARTESIAN_POINT ( 'NONE',  ( -48.11878132662029373, -279.9187897701352199, -194.0651950902481246 ) ) ;
#6544=CARTESIAN_POINT ( 'NONE',  ( 11.47591344234680477, -282.0633261890745871, -329.9497106719672956 ) ) ;
#6545=CARTESIAN_POINT ( 'NONE',  ( -4.911389980194055482, -284.4789127216827183, -202.7209562927560000 ) ) ;
#6546=CARTESIAN_POINT ( 'NONE',  ( 20.29633185581394983, -280.3429185512247273, -317.1649348857197310 ) ) ;
#6547=CARTESIAN_POINT ( 'NONE',  ( -84.24188727825426781, -283.4068543108936638, -211.8344309851138121 ) ) ;
#6548=CARTESIAN_POINT ( 'NONE',  ( -68.37268570619971797, -278.1317639748304487, -200.6347005949525624 ) ) ;
#6549=CARTESIAN_POINT ( 'NONE',  ( 37.42138855115708651, -286.2572660653249272, -253.2155686856430918 ) ) ;
#6550=CARTESIAN_POINT ( 'NONE',  ( -34.04360771932221041, -274.8975283699658121, -197.2740171113412089 ) ) ;
#6552=CARTESIAN_POINT ( 'NONE',  ( -86.47668379385717685, -292.9567183766341145, -215.2269578464480446 ) ) ;
#6553=CARTESIAN_POINT ( 'NONE',  ( -5.377410422757828101, -275.8898087487230555, -200.9572961958038775 ) ) ;
#6554=CARTESIAN_POINT ( 'NONE',  ( -107.1380903662694379, -277.9326703360477495, -291.9909291711151695 ) ) ;
#6555=CARTESIAN_POINT ( 'NONE',  ( -97.46489713158233315, -291.3632090535338648, -222.2549729840611406 ) ) ;
#6557=CARTESIAN_POINT ( 'NONE',  ( 38.17975426672617800, -279.6627535129732109, -272.7744396278453678 ) ) ;
#6558=CARTESIAN_POINT ( 'NONE',  ( -84.26466945018242427, -291.2603840285428873, -209.2428341877914022 ) ) ;
#6559=CARTESIAN_POINT ( 'NONE',  ( -79.65691922584757378, -290.5235712626206919, -210.5258054354374906 ) ) ;
#6561=CARTESIAN_POINT ( 'NONE',  ( 12.05883123497936893, -292.3655376327747035, -326.8621103334050986 ) ) ;
#6565=CARTESIAN_POINT ( 'NONE',  ( 24.90358327567604846, -292.5317611427775546, -232.0091707885733854 ) ) ;
#6567=CARTESIAN_POINT ( 'NONE',  ( -67.74223827176246004, -274.9809262143061233, -333.4151289067050357 ) ) ;
#6568=CARTESIAN_POINT ( 'NONE',  ( -114.1025628679917645, -295.6205387770629045, -269.5928968527447296 ) ) ;
#6570=CARTESIAN_POINT ( 'NONE',  ( -113.4117338338399605, -285.7645654467869463, -278.5249555656179155 ) ) ;
#6571=CARTESIAN_POINT ( 'NONE',  ( -37.27874143033333354, -285.8862449826743273, -197.3487066273611958 ) ) ;
#6573=CARTESIAN_POINT ( 'NONE',  ( 34.26479472108430002, -277.3004929461735060, -287.8274800447115354 ) ) ;
#6574=CARTESIAN_POINT ( 'NONE',  ( -35.63778818994382647, -293.0508104871523187, -344.9992501454398166 ) ) ;
#6575=CARTESIAN_POINT ( 'NONE',  ( -66.43104666926203095, -297.1985343367881001, -338.4183287162916827 ) ) ;
#6576=CARTESIAN_POINT ( 'NONE',  ( 35.74802914649394125, -274.4351054550053846, -277.0709599166363546 ) ) ;
#6579=CARTESIAN_POINT ( 'NONE',  ( -109.4192376298144609, -295.8751840822670260, -297.5406420609234033 ) ) ;
#6580=CARTESIAN_POINT ( 'NONE',  ( -5.147955647059831996, -290.5451969658647045, -337.4794986122409455 ) ) ;
#6581=CARTESIAN_POINT ( 'NONE',  ( -70.45673859265708927, -295.6154843447001213, -203.0537799537354147 ) ) ;
#6582=CARTESIAN_POINT ( 'NONE',  ( 8.049715046464978485, -289.0638573547333863, -327.6630559626719332 ) ) ;
#6584=CARTESIAN_POINT ( 'NONE',  ( -17.04263941731080934, -279.3667908485597877, -196.3289064352503885 ) ) ;
#6585=CARTESIAN_POINT ( 'NONE',  ( -4.538476584350812360, -295.2826329961549732, -339.9259923751421297 ) ) ;
#6586=CARTESIAN_POINT ( 'NONE',  ( -88.67231831860898694, -287.9030610804585990, -326.0878899559325532 ) ) ;
#6587=CARTESIAN_POINT ( 'NONE',  ( -65.59178689926186223, -295.7448866879855700, -341.9831347632746770 ) ) ;
#6588=CARTESIAN_POINT ( 'NONE',  ( 17.99122801174845421, -294.5640015850973441, -318.0284220055924607 ) ) ;
#6593=CARTESIAN_POINT ( 'NONE',  ( -38.88655491756519211, -290.5913193115104605, -346.6521474590123830 ) ) ;
#6594=CARTESIAN_POINT ( 'NONE',  ( -111.2586520408596868, -294.4809262143061801, -234.7283546768995564 ) ) ;
#6595=CARTESIAN_POINT ( 'NONE',  ( -74.95083019618745368, -278.9133656202303087, -203.2875306161356832 ) ) ;
#6596=CARTESIAN_POINT ( 'NONE',  ( -33.37417773616327565, -285.0022726105054858, -345.1020945705409986 ) ) ;
#6597=CARTESIAN_POINT ( 'NONE',  ( -35.14683484195653307, -284.6539052169579804, -193.9688316563729984 ) ) ;
#6598=CARTESIAN_POINT ( 'NONE',  ( -71.86183079828371945, -287.5919262509218584, -336.3275854164556904 ) ) ;
#6599=CARTESIAN_POINT ( 'NONE',  ( 29.46527736692121380, -277.8832283038901210, -306.2089579011853857 ) ) ;
#6602=CARTESIAN_POINT ( 'NONE',  ( -105.5142875194777332, -278.9024818493712132, -244.1140122844505811 ) ) ;
#6603=CARTESIAN_POINT ( 'NONE',  ( -108.9854890862335424, -278.0929445793325385, -255.7703834221395880 ) ) ;
#6604=CARTESIAN_POINT ( 'NONE',  ( -0.2072120995418920142, -275.6137855762760296, -203.2453493493229928 ) ) ;
#6605=CARTESIAN_POINT ( 'NONE',  ( -108.1397975735866055, -277.7207934531446085, -241.1098254350427226 ) ) ;
#6606=CARTESIAN_POINT ( 'NONE',  ( -107.6144582921256045, -259.8900720772599016, -316.0350854841208275 ) ) ;
#6607=CARTESIAN_POINT ( 'NONE',  ( -105.4058824157608285, -273.9540124396383476, -234.7484878119597624 ) ) ;
#6608=CARTESIAN_POINT ( 'NONE',  ( -84.86424733187504899, -298.8364794797370223, -210.5262301783543535 ) ) ;
#6609=CARTESIAN_POINT ( 'NONE',  ( -85.33152481854864391, -281.9090924074130839, -210.2361428286349110 ) ) ;
#6610=DIRECTION ( 'NONE',  ( 0.000000000000000000, 0.000000000000000000, 1.000000000000000000 ) ) ;
#6611=CARTESIAN_POINT ( 'NONE',  ( -30.51613812302811723, -287.2200231353003232, -197.3194357045243805 ) ) ;
#6612=CARTESIAN_POINT ( 'NONE',  ( -3.955078835683296656, -288.2465432557098097, -202.0876632292296051 ) ) ;
#6613=CARTESIAN_POINT ( 'NONE',  ( 31.49259726753807342, -287.2279810332042302, -294.9727447088218923 ) ) ;
#6614=CARTESIAN_POINT ( 'NONE',  ( -108.9688924601785658, -284.4178006332363680, -242.1258312062719824 ) ) ;
#6615=CARTESIAN_POINT ( 'NONE',  ( 32.74269016030901724, -279.6465110759282311, -247.0780914409574507 ) ) ;
#6616=CARTESIAN_POINT ( 'NONE',  ( -65.58474050235567177, -287.5394273996338370, -201.6536694010913777 ) ) ;
#6617=CARTESIAN_POINT ( 'NONE',  ( 22.68942733861521432, -279.4405852020823318, -227.6180309575036631 ) ) ;
#6618=CARTESIAN_POINT ( 'NONE',  ( -36.44345521342935967, -278.3558744321240965, -343.8613323765147811 ) ) ;
#6619=CARTESIAN_POINT ( 'NONE',  ( 33.89235839777776249, -275.8298007282705839, -254.0664438122052786 ) ) ;
#6620=CARTESIAN_POINT ( 'NONE',  ( -20.59821986002108574, -287.6368400893687181, -345.1661836310428271 ) ) ;
#6621=CARTESIAN_POINT ( 'NONE',  ( 24.98231923505507979, -282.9523804796303352, -315.3264808893650297 ) ) ;
#6622=CARTESIAN_POINT ( 'NONE',  ( -100.9491547924593959, -285.6168232319852791, -226.9816782593109963 ) ) ;
#6623=CARTESIAN_POINT ( 'NONE',  ( 13.33357447749409985, -280.9515796475541833, -217.7453004786957536 ) ) ;
#6626=PLANE ( 'NONE',  #89647 ) ;
#6627=CARTESIAN_POINT ( 'NONE',  ( 19.65950247315573307, -290.0989604033294995, -320.2922761551112103 ) ) ;
#6629=CARTESIAN_POINT ( 'NONE',  ( -112.4376616308706929, -289.4219280805659196, -255.6678028095986690 ) ) ;
#6630=CARTESIAN_POINT ( 'NONE',  ( -78.97902877870349414, -272.5344233526247422, -210.0521894456521466 ) ) ;
#6631=CARTESIAN_POINT ( 'NONE',  ( 11.12762384311921515, -293.7499935276551355, -330.1292918364587194 ) ) ;
#6632=CARTESIAN_POINT ( 'NONE',  ( -110.6607769990965977, -289.1289535525201586, -262.9435227937988770 ) ) ;
#6633=CARTESIAN_POINT ( 'NONE',  ( 33.60681202856758887, -291.5147991502217906, -249.1063127810191702 ) ) ;
#6634=CARTESIAN_POINT ( 'NONE',  ( -5.606931943497451165, -289.8302344199476011, -336.5429507958160116 ) ) ;
#6635=CARTESIAN_POINT ( 'NONE',  ( -54.49178911615187815, -288.3376638359845856, -195.3683826091709363 ) ) ;
#6637=CARTESIAN_POINT ( 'NONE',  ( -0.2471318021208591398, -290.5593828569722064, -335.6041203877783232 ) ) ;
#6638=CARTESIAN_POINT ( 'NONE',  ( -68.83131466645507146, -289.6390286043416609, -202.0944082800476167 ) ) ;
#6639=CARTESIAN_POINT ( 'NONE',  ( -95.33902107660433956, -293.2081158090055055, -222.7880995410212108 ) ) ;
#6640=CARTESIAN_POINT ( 'NONE',  ( -87.07987596438424305, -284.7063310625655390, -324.1847639097438787 ) ) ;
#6641=CARTESIAN_POINT ( 'NONE',  ( 19.89742046132858633, -294.8791675456744201, -221.6207126353536125 ) ) ;
#6645=CARTESIAN_POINT ( 'NONE',  ( -91.99693719222734956, -275.2566046300505036, -218.4653892081879007 ) ) ;
#6646=CARTESIAN_POINT ( 'NONE',  ( -1.181068500683291056, -281.7562840504023143, -333.9615145806608894 ) ) ;
#6647=CARTESIAN_POINT ( 'NONE',  ( -34.80369346456757285, -281.0201362912669083, -345.3309444503383361 ) ) ;
#6648=CARTESIAN_POINT ( 'NONE',  ( -112.7282654981038377, -295.9364926349201710, -255.4266029986495425 ) ) ;
#6649=CARTESIAN_POINT ( 'NONE',  ( 30.01745664834820104, -273.3826950467091592, -239.5659295888317786 ) ) ;
#6650=CARTESIAN_POINT ( 'NONE',  ( -110.2936654037478093, -276.8244089385058260, -255.4875862541763922 ) ) ;
#6651=CARTESIAN_POINT ( 'NONE',  ( -109.6241325977257901, -297.6923411541915812, -283.7158304978031538 ) ) ;
#6654=CARTESIAN_POINT ( 'NONE',  ( -103.2881996614228086, -297.5369145434791562, -303.1325174747352094 ) ) ;
#6655=LINE ( 'NONE', #36448, #79231 ) ;
#6656=CARTESIAN_POINT ( 'NONE',  ( -92.87363088870235117, -298.0317174063097241, -222.7098557073385621 ) ) ;
#6658=CARTESIAN_POINT ( 'NONE',  ( -13.20614202235572776, -284.3842513691508884, -198.9756738344607356 ) ) ;
#6659=CARTESIAN_POINT ( 'NONE',  ( -93.77702672893708780, -273.0415946126373683, -224.0376431982256804 ) ) ;
#6661=CARTESIAN_POINT ( 'NONE',  ( -71.06623095477689844, -285.6193044007573008, -201.1393293570176297 ) ) ;
#6662=CARTESIAN_POINT ( 'NONE',  ( 30.34207597361525544, -287.6946251363839906, -307.1420669386396298 ) ) ;
#6663=CARTESIAN_POINT ( 'NONE',  ( -112.5896905899195843, -298.4694656633264458, -275.2581577672503954 ) ) ;
#6664=CARTESIAN_POINT ( 'NONE',  ( 29.12632607952265573, -291.0959216673146557, -235.9804560406519158 ) ) ;
#6665=CARTESIAN_POINT ( 'NONE',  ( -17.02482706760614661, -279.5051879767985383, -196.2572483867477331 ) ) ;
#6666=CARTESIAN_POINT ( 'NONE',  ( -69.91165696735023971, -286.9809262143061801, -337.9199732462171255 ) ) ;
#6668=AXIS2_PLACEMENT_3D ( 'NONE', #19350, #48212, #77115 ) ;
#6669=CARTESIAN_POINT ( 'NONE',  ( -10.59103117119208370, -285.2039481218492938, -201.9989092317847224 ) ) ;
#6671=CARTESIAN_POINT ( 'NONE',  ( -96.54461299498061067, -287.9203992070815730, -316.4255057361012291 ) ) ;
#6672=CARTESIAN_POINT ( 'NONE',  ( -93.45417681046285452, -274.7455148904640509, -222.5703260860421722 ) ) ;
#6673=CARTESIAN_POINT ( 'NONE',  ( -77.20076106695164242, -280.9545562995942873, -205.1088946031197224 ) ) ;
#6674=CARTESIAN_POINT ( 'NONE',  ( -101.7236804649435840, -294.0498093946732752, -309.5193535032951218 ) ) ;
#6675=CARTESIAN_POINT ( 'NONE',  ( 33.76038918893654994, -281.3339898320557495, -253.8234973932851801 ) ) ;
#6676=CARTESIAN_POINT ( 'NONE',  ( -99.09371044264601380, -297.3308483736353196, -224.3424893930035466 ) ) ;
#6677=CARTESIAN_POINT ( 'NONE',  ( -68.35680922567161133, -299.1573103713457726, -203.4984573578359175 ) ) ;
#6678=CARTESIAN_POINT ( 'NONE',  ( 13.30024417629429756, -284.8332986952365786, -214.2132067574345058 ) ) ;
#6679=CARTESIAN_POINT ( 'NONE',  ( 13.77899791739798196, -282.7684531203459528, -215.4114174452151929 ) ) ;
#6680=CARTESIAN_POINT ( 'NONE',  ( -103.9275401027235830, -296.0222580210623846, -239.7475550269165581 ) ) ;
#6683=CARTESIAN_POINT ( 'NONE',  ( -59.41090076414670307, -285.3190492716215090, -341.7232149109100305 ) ) ;
#6684=DIRECTION ( 'NONE',  ( 0.9951408606192333473, 1.205805641958531838E-17, 0.09846150276129089773 ) ) ;
#6685=CARTESIAN_POINT ( 'NONE',  ( -110.4683760289727132, -287.8380690714490129, -287.0191576251351080 ) ) ;
#6686=CARTESIAN_POINT ( 'NONE',  ( 37.07979331617996621, -274.9891136004775376, -289.4817909455644553 ) ) ;
#6689=CARTESIAN_POINT ( 'NONE',  ( -0.08912516867963633793, -292.3961869890320600, -207.5817769267703454 ) ) ;
#6690=CARTESIAN_POINT ( 'NONE',  ( 7.549496466245935622, -282.1970928417822506, -211.8543871336078155 ) ) ;
#6691=CARTESIAN_POINT ( 'NONE',  ( 29.89137663140893864, -277.5579937415433847, -300.7938931191723100 ) ) ;
#6692=CARTESIAN_POINT ( 'NONE',  ( -55.54409579114047801, -284.7072420986251586, -344.5721621971557056 ) ) ;
#6693=CARTESIAN_POINT ( 'NONE',  ( 8.027426942944480004, -281.2113236907149485, -328.1215350966822371 ) ) ;
#6694=CARTESIAN_POINT ( 'NONE',  ( -109.5506168704054204, -280.8136479806623811, -250.0434573790394381 ) ) ;
#6695=CARTESIAN_POINT ( 'NONE',  ( -43.28975629721916363, -297.9791363799269561, -193.5379876853039889 ) ) ;
#6696=CARTESIAN_POINT ( 'NONE',  ( 8.239354767634775811, -276.2813582099733480, -332.4865172601004701 ) ) ;
#6697=CARTESIAN_POINT ( 'NONE',  ( 20.44854402476903488, -294.8210435425579590, -223.4197359779784904 ) ) ;
#6699=CARTESIAN_POINT ( 'NONE',  ( 82.64890176555634582, -299.5541904835127980, -192.9651424135224147 ) ) ;
#6700=CARTESIAN_POINT ( 'NONE',  ( -110.7773829546874538, -294.4540764799666590, -289.0550716743179009 ) ) ;
#6701=CARTESIAN_POINT ( 'NONE',  ( -68.30295365371935645, -273.1418429257196863, -204.1704551858708214 ) ) ;
#6703=CARTESIAN_POINT ( 'NONE',  ( -16.67587515589574565, -296.3101544459350976, -343.8708198234176621 ) ) ;
#6704=CARTESIAN_POINT ( 'NONE',  ( 21.98888790928170067, -295.4111832956580201, -318.8367466605033655 ) ) ;
#6705=CARTESIAN_POINT ( 'NONE',  ( -28.94268546668699216, -290.9455890379921925, -344.7216248270497090 ) ) ;
#6706=CARTESIAN_POINT ( 'NONE',  ( -46.14851910969489523, -275.1638176593491494, -344.7263281219547935 ) ) ;
#6708=CARTESIAN_POINT ( 'NONE',  ( -98.04609444020337605, -279.8820406440989359, -313.4679384391710073 ) ) ;
#6709=CARTESIAN_POINT ( 'NONE',  ( -111.6809736828326720, -294.5819116204035026, -274.2323713548228739 ) ) ;
#6710=CARTESIAN_POINT ( 'NONE',  ( 34.44646749587986534, -283.7245050397887667, -294.7475342079135885 ) ) ;
#6711=CARTESIAN_POINT ( 'NONE',  ( -27.78268987509830268, -285.0967239093956209, -197.6778916086147433 ) ) ;
#6712=CARTESIAN_POINT ( 'NONE',  ( 123.4450140854237645, 148.1040090397345352, -262.7932479617338117 ) ) ;
#6714=CARTESIAN_POINT ( 'NONE',  ( -108.0480724537290058, -284.4595844093128676, -252.1211508938320662 ) ) ;
#6715=CARTESIAN_POINT ( 'NONE',  ( 1.206655381343710864, -281.6335901744072885, -204.0019679940370736 ) ) ;
#6716=CARTESIAN_POINT ( 'NONE',  ( -109.8537878895348285, -283.0342814121304400, -295.0594144146552367 ) ) ;
#6718=CARTESIAN_POINT ( 'NONE',  ( -72.41004682434640927, -280.5408137560759769, -202.0601189151636277 ) ) ;
#6719=CARTESIAN_POINT ( 'NONE',  ( -105.7154506062859411, -279.6315352972225128, -304.3582219816107113 ) ) ;
#6720=CARTESIAN_POINT ( 'NONE',  ( -82.08285599513421005, -276.9094976428775681, -214.2051214447836571 ) ) ;
#6721=CARTESIAN_POINT ( 'NONE',  ( 66.05521907569730899, 47.24546878876408584, -318.8896612879527197 ) ) ;
#6723=CARTESIAN_POINT ( 'NONE',  ( -76.26993376521713230, -299.5323573760761064, -206.1947854090703061 ) ) ;
#6725=CARTESIAN_POINT ( 'NONE',  ( -71.67628606350481846, -277.6163352684956180, -204.0671329830324794 ) ) ;
#6726=CARTESIAN_POINT ( 'NONE',  ( -69.21877995007181994, -293.3987208059937757, -201.3699690410987557 ) ) ;
#6727=CARTESIAN_POINT ( 'NONE',  ( 23.01246486512854972, -293.4749351197648366, -311.6960472579104362 ) ) ;
#6728=CARTESIAN_POINT ( 'NONE',  ( -110.7250515336934740, -289.7671005403453250, -293.6525386480440716 ) ) ;
#6729=CARTESIAN_POINT ( 'NONE',  ( -13.97958449701159900, -293.3295739833139351, -343.1128729099827410 ) ) ;
#6730=CARTESIAN_POINT ( 'NONE',  ( -24.98806372102210460, -284.6120460767558598, -197.5505584061987463 ) ) ;
#6731=CARTESIAN_POINT ( 'NONE',  ( 7.402194449093554951, -294.5301292013162424, -211.1255764927018106 ) ) ;
#6732=CARTESIAN_POINT ( 'NONE',  ( 29.77159426834535694, -283.2694102619713021, -300.4369155396558995 ) ) ;
#6734=CARTESIAN_POINT ( 'NONE',  ( -113.7737673442578625, -291.5898537722490005, -262.6724811960321517 ) ) ;
#6735=CARTESIAN_POINT ( 'NONE',  ( -43.76274118921946865, -280.4613092305531836, -197.5320077233581060 ) ) ;
#6736=CARTESIAN_POINT ( 'NONE',  ( -2.163559205135533237, -293.3918340353606595, -338.4089476390099094 ) ) ;
#6738=CARTESIAN_POINT ( 'NONE',  ( 0.6483754924009604848, -289.3622482158037315, -337.2113146170569280 ) ) ;
#6739=CARTESIAN_POINT ( 'NONE',  ( -34.66268009850591625, -289.5116761196070456, -347.2529234958047937 ) ) ;
#6740=CARTESIAN_POINT ( 'NONE',  ( 13.13802065155954324, -286.9480231644328114, -217.5581098758366920 ) ) ;
#6743=CARTESIAN_POINT ( 'NONE',  ( -47.44306142105438795, -297.0396529500850988, -345.4495190763924484 ) ) ;
#6744=CARTESIAN_POINT ( 'NONE',  ( -62.66591989841295884, -296.4141373707665821, -198.1670589112384846 ) ) ;
#6745=CARTESIAN_POINT ( 'NONE',  ( -110.4040180262971660, -277.5356249193470717, -276.0853772726320585 ) ) ;
#6746=CARTESIAN_POINT ( 'NONE',  ( -81.21014955545675207, -272.9814238445582077, -207.0898685236535641 ) ) ;
#6747=CARTESIAN_POINT ( 'NONE',  ( -34.29169290404533399, -293.4929862397166289, -343.9913102248517021 ) ) ;
#6748=CARTESIAN_POINT ( 'NONE',  ( 5.748759157823479349, -276.4048141683725817, -210.1214935816987293 ) ) ;
#6749=CARTESIAN_POINT ( 'NONE',  ( -105.5046300928302259, -271.0818495909373951, -240.8254948327308114 ) ) ;
#6750=CARTESIAN_POINT ( 'NONE',  ( 32.17217576012168934, -294.4440418615810131, -246.6455947132782285 ) ) ;
#6751=CARTESIAN_POINT ( 'NONE',  ( -105.2430635470345521, -297.2632115875783256, -297.9949906519991600 ) ) ;
#6753=CARTESIAN_POINT ( 'NONE',  ( -105.5145906721402582, -294.1369017818259408, -302.0231681110018371 ) ) ;
#6754=CARTESIAN_POINT ( 'NONE',  ( -48.96278628175142700, -298.5593706151875040, -194.2926344110418029 ) ) ;
#6755=CARTESIAN_POINT ( 'NONE',  ( 26.19570646661878754, -286.6336026538934334, -307.5882615394839945 ) ) ;
#6756=CARTESIAN_POINT ( 'NONE',  ( -109.1178196114578043, -274.8347243191913094, -248.4300993436286547 ) ) ;
#6757=CARTESIAN_POINT ( 'NONE',  ( -111.7603764912722113, -273.2914829440908306, -250.6280109516932839 ) ) ;
#6758=CARTESIAN_POINT ( 'NONE',  ( -101.4838653887274518, -296.4092326601953573, -305.2591139474765214 ) ) ;
#6759=CARTESIAN_POINT ( 'NONE',  ( -110.4953971236689938, -280.7637905563339018, -252.2265270257778695 ) ) ;
#6760=CARTESIAN_POINT ( 'NONE',  ( -28.26676924479576414, -278.8497063325251020, -194.3411066717031872 ) ) ;
#6761=CARTESIAN_POINT ( 'NONE',  ( -79.11132393653237216, -282.9484398959698410, -334.9259018302595905 ) ) ;
#6762=CARTESIAN_POINT ( 'NONE',  ( 36.78514330758493145, -275.1579199981619581, -290.8680523908661826 ) ) ;
#6763=CARTESIAN_POINT ( 'NONE',  ( -9.138071579272676104, -278.8147377829336619, -199.5727308531745621 ) ) ;
#6764=CARTESIAN_POINT ( 'NONE',  ( -42.28346906920241111, -277.9898048292583326, -195.3570691104125103 ) ) ;
#6765=CARTESIAN_POINT ( 'NONE',  ( -110.9302533213375170, -271.1630414604915700, -267.5971677107045252 ) ) ;
#6766=CARTESIAN_POINT ( 'NONE',  ( 30.76387501785565348, -277.9662554485501573, -301.8941007075530365 ) ) ;
#6768=CARTESIAN_POINT ( 'NONE',  ( 14.32908211502242857, -290.7937678050400336, -215.4393165220135131 ) ) ;
#6769=CARTESIAN_POINT ( 'NONE',  ( -72.17226653832392458, -291.6043158448395616, -201.6746056895983941 ) ) ;
#6770=CARTESIAN_POINT ( 'NONE',  ( 13.65843380474318991, -278.3402571758993531, -325.6498661402596326 ) ) ;
#6771=CARTESIAN_POINT ( 'NONE',  ( 10.78751916717431314, -272.7169704748302479, -212.7728417827638623 ) ) ;
#6772=DIRECTION ( 'NONE',  ( 0.000000000000000000, 0.000000000000000000, -1.000000000000000000 ) ) ;
#6774=CARTESIAN_POINT ( 'NONE',  ( -105.0402076491763808, -282.9781974211392139, -237.9633363029016664 ) ) ;
#6776=CARTESIAN_POINT ( 'NONE',  ( 32.72129114376627967, -292.6353244162791043, -292.2313662452424978 ) ) ;
#6777=CARTESIAN_POINT ( 'NONE',  ( 36.78760162229094277, -285.6290532716450912, -265.5295249872702357 ) ) ;
#6780=CARTESIAN_POINT ( 'NONE',  ( -41.16599750196969154, -293.1001064511826257, -345.2764686778536998 ) ) ;
#6781=CARTESIAN_POINT ( 'NONE',  ( -113.4586947301442450, -283.1087249867977107, -264.2840055189940358 ) ) ;
#6782=CARTESIAN_POINT ( 'NONE',  ( -109.0719931358301977, -280.3787816277598495, -253.0058455138177180 ) ) ;
#6783=CARTESIAN_POINT ( 'NONE',  ( -57.66543618221821532, -287.0006128014463229, -196.4483851348814483 ) ) ;
#6784=CARTESIAN_POINT ( 'NONE',  ( -19.96586882316425360, -278.5122215547523865, -196.3337278217716175 ) ) ;
#6785=CARTESIAN_POINT ( 'NONE',  ( 21.99157979706356869, -286.9567232072396905, -227.7487042747412147 ) ) ;
#6787=CARTESIAN_POINT ( 'NONE',  ( -73.11267154320242412, -278.9614349638636668, -334.6858972757340212 ) ) ;
#6788=CARTESIAN_POINT ( 'NONE',  ( -110.5534815158028294, -279.3512023371334294, -270.6488695304282714 ) ) ;
#6790=CARTESIAN_POINT ( 'NONE',  ( -43.55631160385355827, -287.9540348119309670, -195.2104912067817963 ) ) ;
#6792=CARTESIAN_POINT ( 'NONE',  ( -108.8878111973532157, -296.7481459817725522, -241.7546394066846744 ) ) ;
#6793=CARTESIAN_POINT ( 'NONE',  ( 24.89449991426167230, -290.0915546015717723, -311.5973648834024630 ) ) ;
#6795=CARTESIAN_POINT ( 'NONE',  ( -119.3990491898856732, -281.0519495502701943, -270.3937649182068412 ) ) ;
#6797=CARTESIAN_POINT ( 'NONE',  ( -65.51583670687578831, -271.6845087381012149, -200.6605136050853844 ) ) ;
#6799=CARTESIAN_POINT ( 'NONE',  ( 1.345532328506472419, -292.9441950195819118, -336.0097162928116745 ) ) ;
#6800=CARTESIAN_POINT ( 'NONE',  ( -53.16881202234307580, -294.7681172037196120, -341.7397970965650416 ) ) ;
#6801=CARTESIAN_POINT ( 'NONE',  ( -11.79965379505463297, -287.9109661624901833, -201.2357852788498462 ) ) ;
#6802=AXIS2_PLACEMENT_3D ( 'NONE', #82364, #1898, #46365 ) ;
#6803=CARTESIAN_POINT ( 'NONE',  ( 19.60156281330873540, -282.6506941180336412, -223.0610284341442480 ) ) ;
#6804=CARTESIAN_POINT ( 'NONE',  ( -7.136018920196121940, -290.0888730158718545, -340.5623089576561711 ) ) ;
#6805=CARTESIAN_POINT ( 'NONE',  ( -97.75979101718108666, -291.2364365761283693, -317.2967395087235900 ) ) ;
#6806=CARTESIAN_POINT ( 'NONE',  ( -43.06068304860170315, -285.1243805312324184, -345.1942184142553742 ) ) ;
#6807=CARTESIAN_POINT ( 'NONE',  ( -93.33253387578001536, -277.9963940603283845, -323.2961784113347221 ) ) ;
#6808=CARTESIAN_POINT ( 'NONE',  ( 34.98405915197686511, -291.9137872170805394, -292.4082077718963433 ) ) ;
#6809=CARTESIAN_POINT ( 'NONE',  ( -14.22573591802529513, -280.1770498845876318, -196.8569211956442189 ) ) ;
#6810=CARTESIAN_POINT ( 'NONE',  ( -68.82767353928764464, -275.4942247610514414, -203.1199678787864684 ) ) ;
#6811=CARTESIAN_POINT ( 'NONE',  ( -20.25526795762937127, -288.7662352645560304, -195.3538533559490702 ) ) ;
#6812=CARTESIAN_POINT ( 'NONE',  ( 36.30865968177557335, -273.5549337528162823, -251.6635642317122006 ) ) ;
#6814=CARTESIAN_POINT ( 'NONE',  ( -46.45792522568929428, -279.4411332258046059, -197.8194021589485203 ) ) ;
#6815=CARTESIAN_POINT ( 'NONE',  ( 23.21363838431332738, -277.3871158940817736, -317.2978494860217893 ) ) ;
#6816=CARTESIAN_POINT ( 'NONE',  ( -103.0667027729937359, -298.4244180156493940, -237.1477701089136758 ) ) ;
#6817=CARTESIAN_POINT ( 'NONE',  ( -111.9931577696146121, -283.3858076672752304, -288.3047849279770389 ) ) ;
#6818=CARTESIAN_POINT ( 'NONE',  ( -109.7059863760641463, -292.5144412789284729, -254.8245774364963268 ) ) ;
#6819=CARTESIAN_POINT ( 'NONE',  ( -112.7556112951421596, -274.2948001941855978, -259.0834997254065115 ) ) ;
#6820=CARTESIAN_POINT ( 'NONE',  ( -113.6901519526754072, -273.9388369354260817, -264.6796541390648372 ) ) ;
#6821=CARTESIAN_POINT ( 'NONE',  ( -3.484979095569499918, -296.6043879013998890, -337.1118981292720491 ) ) ;
#6822=CARTESIAN_POINT ( 'NONE',  ( -83.95613797422839752, -281.6935959865587620, -328.9692612425107541 ) ) ;
#6823=CARTESIAN_POINT ( 'NONE',  ( -107.2394501601043402, -290.6329687966003803, -237.9843448037091491 ) ) ;
#6824=CARTESIAN_POINT ( 'NONE',  ( 14.86406471174902499, -274.3325507775545020, -323.7847882684168894 ) ) ;
#6825=CARTESIAN_POINT ( 'NONE',  ( -15.66079108021488331, -287.9281089825261688, -197.2557854055254438 ) ) ;
#6826=CARTESIAN_POINT ( 'NONE',  ( -98.55008013413456069, -290.0307759435599451, -229.9234233872433038 ) ) ;
#6828=CARTESIAN_POINT ( 'NONE',  ( -110.2253551251877326, -288.8343259320022298, -293.4814212516201906 ) ) ;
#6829=CARTESIAN_POINT ( 'NONE',  ( -109.7204949041569790, -290.3512635300337479, -260.3220032173885556 ) ) ;
#6831=CARTESIAN_POINT ( 'NONE',  ( 36.09339810295367101, -288.9109374044105039, -292.5150998761214396 ) ) ;
#6832=CARTESIAN_POINT ( 'NONE',  ( -48.60691564909392071, -277.5326890548631695, -342.5594715398640346 ) ) ;
#6833=CARTESIAN_POINT ( 'NONE',  ( -53.23865245455921524, -294.1715945164720551, -345.4406361985554099 ) ) ;
#6834=CARTESIAN_POINT ( 'NONE',  ( -41.55524485777256416, -283.7551821413716198, -347.1959179724448745 ) ) ;
#6835=CARTESIAN_POINT ( 'NONE',  ( -112.9782761821414283, -285.0679061440110900, -255.7710135701557590 ) ) ;
#6836=CARTESIAN_POINT ( 'NONE',  ( 11.31675292249747855, -281.0823067329237119, -215.9144244794644578 ) ) ;
#6837=CARTESIAN_POINT ( 'NONE',  ( 194.1796378510228749, 279.1575638736977112, -125.9076664125385037 ) ) ;
#6838=CARTESIAN_POINT ( 'NONE',  ( -100.6270238236691341, -247.1647810672108676, -333.6273736269536130 ) ) ;
#6839=CARTESIAN_POINT ( 'NONE',  ( -103.7292136647523222, -253.6277699525920752, -324.3870440700492850 ) ) ;
#6840=CARTESIAN_POINT ( 'NONE',  ( -106.4555858548876159, -272.0677620063422069, -246.3637738258152865 ) ) ;
#6841=CARTESIAN_POINT ( 'NONE',  ( 33.81251353248127600, -274.2406337770659661, -252.7173102048476778 ) ) ;
#6842=CARTESIAN_POINT ( 'NONE',  ( -99.96207412128785563, -295.4662012159903384, -315.1522681502689807 ) ) ;
#6843=CARTESIAN_POINT ( 'NONE',  ( 103.9790695402631542, 114.2035196735941014, -279.8796163930391003 ) ) ;
#6844=CARTESIAN_POINT ( 'NONE',  ( -69.90654276699919478, -272.3170824185372112, -201.1165352077644570 ) ) ;
#6845=CARTESIAN_POINT ( 'NONE',  ( -92.78289610387243158, -299.1067106019873449, -220.9937272232280350 ) ) ;
#6846=CARTESIAN_POINT ( 'NONE',  ( 26.13035353343015998, -289.3736076648922904, -307.5095966231827447 ) ) ;
#6847=CARTESIAN_POINT ( 'NONE',  ( -109.0156728521508143, -291.8340815830548536, -254.9641147490587798 ) ) ;
#6849=CARTESIAN_POINT ( 'NONE',  ( -62.77841576719750094, -298.6701996495469302, -197.9332662254898878 ) ) ;
#6850=CARTESIAN_POINT ( 'NONE',  ( 11.17023993891524292, -287.2377583740539535, -215.6618384412749663 ) ) ;
#6851=CARTESIAN_POINT ( 'NONE',  ( -4.562120616607214352, -295.4340278558877912, -339.8712993806753957 ) ) ;
#6852=CARTESIAN_POINT ( 'NONE',  ( -5.817178022079361632, -295.1410031709812074, -340.5446731036466304 ) ) ;
#6853=CARTESIAN_POINT ( 'NONE',  ( -0.09277589007679333533, -292.7294932912904528, -207.5796107721051555 ) ) ;
#6855=CARTESIAN_POINT ( 'NONE',  ( -13.53971524851210440, -276.2789602045210700, -198.6479412838396001 ) ) ;
#6857=CARTESIAN_POINT ( 'NONE',  ( -93.02488084551742986, -278.7869767283418696, -217.1915935700891112 ) ) ;
#6858=CARTESIAN_POINT ( 'NONE',  ( 30.92249417963552105, -273.5786587781303183, -242.1832972769480250 ) ) ;
#6859=CARTESIAN_POINT ( 'NONE',  ( -109.4362405200949411, -273.8099651867767648, -256.8000895874391745 ) ) ;
#6860=CARTESIAN_POINT ( 'NONE',  ( 35.82134529165360703, -276.4375555199185328, -266.1134143587142944 ) ) ;
#6861=CARTESIAN_POINT ( 'NONE',  ( 11.12193141546653763, -276.4723563065655867, -211.7671220282612978 ) ) ;
#6862=CARTESIAN_POINT ( 'NONE',  ( 31.50655769710617449, -273.9717737252917686, -300.9931958472498650 ) ) ;
#6863=CARTESIAN_POINT ( 'NONE',  ( -109.9046191018525320, -297.0815070544902596, -279.6269827524902780 ) ) ;
#6864=( GEOMETRIC_REPRESENTATION_CONTEXT ( 3 ) GLOBAL_UNCERTAINTY_ASSIGNED_CONTEXT ( ( #83551 ) ) GLOBAL_UNIT_ASSIGNED_CONTEXT ( ( #64964, #56918, #84346 ) ) REPRESENTATION_CONTEXT ( 'NONE', 'WORKASPACE' ) );
#6865=CARTESIAN_POINT ( 'NONE',  ( 16.57862423517864769, -292.8409554647091113, -320.4407898865063089 ) ) ;
#6867=CARTESIAN_POINT ( 'NONE',  ( -112.1138860555012258, -278.8169008992088607, -288.5449083783926767 ) ) ;
#6868=CARTESIAN_POINT ( 'NONE',  ( 34.70750918302831423, -275.8777800387776438, -282.4101755853341729 ) ) ;
#6870=AXIS2_PLACEMENT_3D ( 'NONE', #11708, #3203, #90746 ) ;
#6871=CARTESIAN_POINT ( 'NONE',  ( -18.28854320631695174, -284.9773865967538882, -196.2099722438857157 ) ) ;
#6872=CARTESIAN_POINT ( 'NONE',  ( -81.90466411633786947, -299.4471366281514975, -209.7640378534141519 ) ) ;
#6873=CARTESIAN_POINT ( 'NONE',  ( 82.62449080995027373, -301.4714224534961886, -196.9739619934580048 ) ) ;
#6874=CARTESIAN_POINT ( 'NONE',  ( 23.67437527527419050, -286.1893846156170298, -229.9005749589418031 ) ) ;
#6875=CARTESIAN_POINT ( 'NONE',  ( -93.84954952996797317, -277.4622521423027592, -222.5416621415513418 ) ) ;
#6876=CARTESIAN_POINT ( 'NONE',  ( -79.37669450963343820, -278.0467752045547059, -209.9588484624203772 ) ) ;
#6877=CARTESIAN_POINT ( 'NONE',  ( -55.70587383441166907, -285.2885709944625887, -343.1309728289907639 ) ) ;
#6878=CARTESIAN_POINT ( 'NONE',  ( -68.19041699205519080, -278.6716325336151954, -336.9743919653828925 ) ) ;
#6880=CARTESIAN_POINT ( 'NONE',  ( 35.82353380483935723, -273.6801225773508577, -248.8859689579149688 ) ) ;
#6881=CARTESIAN_POINT ( 'NONE',  ( 34.94120171520702911, -276.0587111588223479, -259.3648184049165479 ) ) ;
#6882=CARTESIAN_POINT ( 'NONE',  ( 36.97803798745025716, -283.4038447058798624, -258.7723949708142186 ) ) ;
#6884=CARTESIAN_POINT ( 'NONE',  ( 37.66428058273490365, -289.5940847440669472, -279.9163628558444543 ) ) ;
#6885=CARTESIAN_POINT ( 'NONE',  ( 18.08390197224154150, -290.8465964040101426, -219.8149839727543906 ) ) ;
#6886=CARTESIAN_POINT ( 'NONE',  ( -6.305593342992922068, -273.1534952555061295, -203.7427754997524971 ) ) ;
#6887=CARTESIAN_POINT ( 'NONE',  ( -11.81356043243047438, -290.5274942293348772, -200.5985058486490118 ) ) ;
#6888=CARTESIAN_POINT ( 'NONE',  ( -90.78337343436103879, -230.3218577325732781, -348.1307343985224634 ) ) ;
#6890=CARTESIAN_POINT ( 'NONE',  ( -104.5544964833918442, -288.5607208999405771, -306.4879467546468277 ) ) ;
#6891=CARTESIAN_POINT ( 'NONE',  ( -13.00673725730827712, -284.6039669252799627, -198.3765113330170209 ) ) ;
#6892=CARTESIAN_POINT ( 'NONE',  ( -3.333066667267752248, -284.0191928491674958, -335.6346259346908596 ) ) ;
#6893=CARTESIAN_POINT ( 'NONE',  ( -99.16201929787168012, -284.8143519411291322, -309.5820160768043934 ) ) ;
#6895=CARTESIAN_POINT ( 'NONE',  ( -55.81059605911486443, -293.7955613790688858, -197.2504656760841328 ) ) ;
#6896=CARTESIAN_POINT ( 'NONE',  ( -35.52854025202275778, -274.4075681216612566, -193.3904917673858677 ) ) ;
#6897=CARTESIAN_POINT ( 'NONE',  ( -95.30249646358021209, -287.9670393870879934, -318.8565526130448688 ) ) ;
#6898=CARTESIAN_POINT ( 'NONE',  ( -22.93890052929812384, -276.8729102018812682, -346.0562929192211072 ) ) ;
#6899=CARTESIAN_POINT ( 'NONE',  ( 35.38352806009255858, -295.7496848076312972, -287.2367871789406877 ) ) ;
#6901=CARTESIAN_POINT ( 'NONE',  ( -83.11486472582501506, -282.3784722272463910, -327.9247881687138033 ) ) ;
#6902=CARTESIAN_POINT ( 'NONE',  ( -56.03294299444257121, -277.8114028498940797, -197.6739637014906066 ) ) ;
#6903=CARTESIAN_POINT ( 'NONE',  ( 7.424657929120416000, -297.0036273313833703, -194.1730573998131888 ) ) ;
#6904=CARTESIAN_POINT ( 'NONE',  ( 31.35470757426955046, -275.2350516737913608, -295.5020920236807456 ) ) ;
#6905=CARTESIAN_POINT ( 'NONE',  ( -12.04017218948744805, -293.9074870923922163, -201.0930043797890221 ) ) ;
#6906=CARTESIAN_POINT ( 'NONE',  ( 35.44216684457012434, -294.6060335039535971, -278.9261934527773974 ) ) ;
#6907=CARTESIAN_POINT ( 'NONE',  ( -37.66994488711937095, -296.3713133498129650, -346.8802599108891513 ) ) ;
#6908=CARTESIAN_POINT ( 'NONE',  ( -86.49154197761680507, -295.5913062068389081, -324.3360478171921955 ) ) ;
#6909=CARTESIAN_POINT ( 'NONE',  ( -97.35373956792248862, -291.9374303022664776, -315.3664915234331261 ) ) ;
#6910=CARTESIAN_POINT ( 'NONE',  ( -83.88151497312459526, -283.8378941471897861, -331.7717632045762457 ) ) ;
#6911=CARTESIAN_POINT ( 'NONE',  ( 4.205934018149265263, -272.7448848494808544, -206.9419376233988999 ) ) ;
#6912=CARTESIAN_POINT ( 'NONE',  ( -2.221011949415980347, -286.3372983410575898, -201.8223747401436867 ) ) ;
#6913=CARTESIAN_POINT ( 'NONE',  ( -18.57971230128489992, -278.7891912710617248, -342.6095408891184775 ) ) ;
#6915=CARTESIAN_POINT ( 'NONE',  ( -87.84813418538628582, -284.3835941454530598, -217.3280286275817730 ) ) ;
#6916=CARTESIAN_POINT ( 'NONE',  ( -3.974031079240675890, -286.6120053661029488, -337.5438045115778323 ) ) ;
#6917=CARTESIAN_POINT ( 'NONE',  ( -104.5266604826868644, -260.4492150524036447, -315.3738353148558531 ) ) ;
#6918=CARTESIAN_POINT ( 'NONE',  ( -4.561334620148513430, -286.0038710971283535, -205.0661252264309553 ) ) ;
#6919=CARTESIAN_POINT ( 'NONE',  ( -37.30230267540845546, -283.9928807237935189, -347.1388402226243670 ) ) ;
#6920=CARTESIAN_POINT ( 'NONE',  ( -57.24149715323748921, -288.3614519093280819, -344.5565880092141242 ) ) ;
#6921=CARTESIAN_POINT ( 'NONE',  ( -102.7356303687088968, -280.6688284196642371, -231.1423127269929978 ) ) ;
#6922=CARTESIAN_POINT ( 'NONE',  ( -112.8099441430402976, -279.7091848142044910, -282.9246532532335436 ) ) ;
#6923=CARTESIAN_POINT ( 'NONE',  ( -49.13981870071936697, -279.7309192988812470, -198.3208209077055528 ) ) ;
#6924=CARTESIAN_POINT ( 'NONE',  ( -43.64561485211081049, -275.9521429260435639, -195.9311257194189579 ) ) ;
#6925=CARTESIAN_POINT ( 'NONE',  ( 29.47564115329079470, -293.0549537924198376, -232.0930777389227444 ) ) ;
#6926=CARTESIAN_POINT ( 'NONE',  ( 20.77864682589926204, -286.2199339869449091, -317.1999061506106159 ) ) ;
#6928=CARTESIAN_POINT ( 'NONE',  ( -88.13157978398666614, -292.9551855496760595, -213.5559374248252595 ) ) ;
#6929=CARTESIAN_POINT ( 'NONE',  ( -109.0787717184319234, -295.6716125633915908, -255.2005293943817037 ) ) ;
#6930=CARTESIAN_POINT ( 'NONE',  ( -4.163817024218998242, -284.5313639721014169, -336.9985119457261931 ) ) ;
#6931=CARTESIAN_POINT ( 'NONE',  ( -80.17060626431941728, -295.3170267777505273, -329.5030851958939593 ) ) ;
#6932=CARTESIAN_POINT ( 'NONE',  ( 39.13179638315010322, -294.5593645940811030, -264.5907765352137062 ) ) ;
#6933=CARTESIAN_POINT ( 'NONE',  ( -7.966087386808290205, -281.0988606643620074, -203.4074090307868516 ) ) ;
#6934=CARTESIAN_POINT ( 'NONE',  ( 37.99016587947605217, -274.4257136689749359, -255.5986596014465135 ) ) ;
#6935=CARTESIAN_POINT ( 'NONE',  ( -38.90976897433122161, -289.7227510883251398, -347.2431961744549085 ) ) ;
#6936=CARTESIAN_POINT ( 'NONE',  ( -11.15161057318202786, -280.8541481673136104, -341.5110442238404858 ) ) ;
#6937=CARTESIAN_POINT ( 'NONE',  ( -114.3689209509520595, -290.8745286872411384, -271.2327552579352528 ) ) ;
#6938=CARTESIAN_POINT ( 'NONE',  ( 28.24861413923276388, -288.3200305144690105, -302.4547024036314156 ) ) ;
#6940=CARTESIAN_POINT ( 'NONE',  ( 166.0114646923310602, 231.9370847612306932, -191.0689560128921300 ) ) ;
#6941=CARTESIAN_POINT ( 'NONE',  ( 103.1691430569825201, 114.4498183994276701, -279.5267493636292784 ) ) ;
#6942=CARTESIAN_POINT ( 'NONE',  ( -37.30987171927208834, -295.5523547857347353, -200.3611179825600459 ) ) ;
#6943=CARTESIAN_POINT ( 'NONE',  ( -96.53033456514194199, -278.3498422243019945, -227.3575450987400757 ) ) ;
#6945=CARTESIAN_POINT ( 'NONE',  ( -22.11684334101605742, -279.1719741586950363, -198.5983022467686965 ) ) ;
#6946=CARTESIAN_POINT ( 'NONE',  ( -35.52003169720737219, -273.7411135690103379, -193.3906927978415240 ) ) ;
#6947=CARTESIAN_POINT ( 'NONE',  ( -53.96950941693697246, -170.4674300608036503, -362.0100880823835041 ) ) ;
#6948=CARTESIAN_POINT ( 'NONE',  ( -69.69623604000952355, -278.2092778345290753, -201.1240814426776637 ) ) ;
#6949=CARTESIAN_POINT ( 'NONE',  ( 13.00798148109448782, -280.3648095250903793, -325.4678903628616808 ) ) ;
#6950=CARTESIAN_POINT ( 'NONE',  ( -100.7170786770327879, -298.8713338101152317, -228.4144446106088537 ) ) ;
#6951=CARTESIAN_POINT ( 'NONE',  ( 24.48267372241567230, -294.5829724668028007, -309.3886089952530938 ) ) ;
#6953=CARTESIAN_POINT ( 'NONE',  ( 1.558507642033911456, -287.2050156837075860, -332.7150858843626224 ) ) ;
#6954=CARTESIAN_POINT ( 'NONE',  ( -34.11578406128840868, -274.7431362305676998, -193.5307447415462434 ) ) ;
#6955=CARTESIAN_POINT ( 'NONE',  ( -52.63716048434380212, -298.0175154456912878, -198.9296210900367896 ) ) ;
#6960=CARTESIAN_POINT ( 'NONE',  ( -35.66947508278408918, -281.1532613951632129, -197.0586240018850503 ) ) ;
#6961=CARTESIAN_POINT ( 'NONE',  ( -35.38488858966578476, -281.8364996814060532, -194.3866839478937720 ) ) ;
#6962=CARTESIAN_POINT ( 'NONE',  ( -90.92175429966927425, -282.8952702857436066, -320.2869253693708060 ) ) ;
#6963=CARTESIAN_POINT ( 'NONE',  ( -72.73920005939122291, -281.4384729274287338, -205.1086660705969109 ) ) ;
#6964=CARTESIAN_POINT ( 'NONE',  ( -5.999160243941402904, -275.1124203219407036, -337.0709891403882921 ) ) ;
#6967=CARTESIAN_POINT ( 'NONE',  ( -6.629830887579506893, -277.4619086557471519, -340.8092852775565689 ) ) ;
#6969=CARTESIAN_POINT ( 'NONE',  ( -99.99286380534586272, -276.5442098938995628, -314.1039800648590585 ) ) ;
#6972=CARTESIAN_POINT ( 'NONE',  ( -91.23930866183877697, -285.7937962642237153, -323.0247163826246037 ) ) ;
#6974=CARTESIAN_POINT ( 'NONE',  ( 33.46706107295545252, -292.5068771936378198, -251.9567417481746077 ) ) ;
#6975=CARTESIAN_POINT ( 'NONE',  ( 36.28539530061574681, -287.1801322140648267, -292.5961028353279403 ) ) ;
#6976=CARTESIAN_POINT ( 'NONE',  ( -19.55086886134803947, -284.5239598567427493, -198.5178139538606956 ) ) ;
#6977=CARTESIAN_POINT ( 'NONE',  ( -110.8977533990320552, -283.1557861643560727, -268.1516061122723613 ) ) ;
#6978=CARTESIAN_POINT ( 'NONE',  ( 16.73624348595687295, -286.5095859844233814, -320.9687456464587285 ) ) ;
#6979=CARTESIAN_POINT ( 'NONE',  ( 29.68329294213124925, -283.1593296971832387, -300.3988542733939653 ) ) ;
#6980=CARTESIAN_POINT ( 'NONE',  ( 22.88933240778906963, -272.9419774280616480, -225.6708128688526358 ) ) ;
#6981=CARTESIAN_POINT ( 'NONE',  ( -103.7301433442240892, -282.4603815668274933, -307.8714469036783612 ) ) ;
#6982=CARTESIAN_POINT ( 'NONE',  ( -64.84571742789454163, -297.4114969671805397, -340.1498183009070999 ) ) ;
#6983=CARTESIAN_POINT ( 'NONE',  ( -96.13021995200431036, -283.1944355199664187, -223.5216221635462830 ) ) ;
#6984=CARTESIAN_POINT ( 'NONE',  ( -87.70109466164885248, -280.2693397686472849, -217.1182879169194564 ) ) ;
#6985=CARTESIAN_POINT ( 'NONE',  ( 35.02642474499729985, -289.8137000907473180, -290.7279003110270423 ) ) ;
#6988=CARTESIAN_POINT ( 'NONE',  ( 25.28540849312504335, -294.9035634149785210, -227.9943107898707240 ) ) ;
#6989=AXIS2_PLACEMENT_3D ( 'NONE', #40541, #2272, #3185 ) ;
#6990=CARTESIAN_POINT ( 'NONE',  ( -82.03096345067650930, -275.6612755223351883, -330.5929234470335132 ) ) ;
#6991=CARTESIAN_POINT ( 'NONE',  ( -105.8554877771612581, -290.1994379943457716, -235.4584931781828061 ) ) ;
#6992=CARTESIAN_POINT ( 'NONE',  ( -26.10548938036544087, -293.3065770096691836, -343.3007367206303115 ) ) ;
#6993=CARTESIAN_POINT ( 'NONE',  ( -91.65002219283027785, -277.9422885543603456, -220.8449627097939469 ) ) ;
#6994=CARTESIAN_POINT ( 'NONE',  ( -91.22235272016261831, -271.3586151295104969, -218.9791671278488536 ) ) ;
#6995=CARTESIAN_POINT ( 'NONE',  ( -7.082400480927849351, -293.7728859642442671, -203.3863595717635349 ) ) ;
#6996=CARTESIAN_POINT ( 'NONE',  ( -54.42813229853332757, -285.7662352645559736, -345.3683826091709648 ) ) ;
#6997=CARTESIAN_POINT ( 'NONE',  ( -33.48937704710156282, -293.4844005883448403, -346.5834846776421045 ) ) ;
#6998=CARTESIAN_POINT ( 'NONE',  ( -37.24675459869111904, -290.6510736777672719, -344.1610597383615868 ) ) ;
#6999=CARTESIAN_POINT ( 'NONE',  ( 27.20361063925697565, -291.2593712531426036, -230.1633094889005520 ) ) ;
#7000=CARTESIAN_POINT ( 'NONE',  ( -78.48896982528417254, -291.0429839221006887, -331.4329218863165920 ) ) ;
#7002=CARTESIAN_POINT ( 'NONE',  ( -109.5769074143431254, -291.2012001682414279, -282.0448711806879487 ) ) ;
#7005=CARTESIAN_POINT ( 'NONE',  ( -102.8840994262729680, -292.2785564555401265, -230.6078038479448082 ) ) ;
#7006=CARTESIAN_POINT ( 'NONE',  ( 37.88539608355938526, -279.6388598177692302, -275.5728101149813938 ) ) ;
#7007=CARTESIAN_POINT ( 'NONE',  ( -85.92902774838911739, -291.3568475447674473, -215.8112333626125974 ) ) ;
#7008=CARTESIAN_POINT ( 'NONE',  ( -91.04645891207493946, -279.6480491895856062, -215.1366148102190152 ) ) ;
#7009=CARTESIAN_POINT ( 'NONE',  ( 36.15678312443506570, -280.9313019580994819, -247.4762485029094137 ) ) ;
#7010=CARTESIAN_POINT ( 'NONE',  ( 31.81558776187212700, -285.1714003761456979, -241.2046241034049103 ) ) ;
#7012=CARTESIAN_POINT ( 'NONE',  ( 23.58522155720736180, -280.2730732385106194, -312.7730938278062922 ) ) ;
#7013=CARTESIAN_POINT ( 'NONE',  ( -111.5057150680691507, -282.6997599146849325, -258.8525272093920648 ) ) ;
#7015=CARTESIAN_POINT ( 'NONE',  ( -112.3113342385274649, -277.2123964157004821, -256.0694552594962943 ) ) ;
#7016=CARTESIAN_POINT ( 'NONE',  ( -111.1975124960409147, -283.2125681013214376, -291.0205344732594313 ) ) ;
#7017=CARTESIAN_POINT ( 'NONE',  ( -96.41779914497033133, -273.9589860196180666, -227.1188957257437835 ) ) ;
#7019=CARTESIAN_POINT ( 'NONE',  ( -98.97880242879470813, -292.7101435435285453, -229.6812116764525911 ) ) ;
#7020=CARTESIAN_POINT ( 'NONE',  ( 13.55834334993410728, -276.1734498998011986, -213.3010256518856522 ) ) ;
#7021=CARTESIAN_POINT ( 'NONE',  ( -9.984379220265084953, -276.3515637505444147, -338.0774528972052622 ) ) ;
#7022=CARTESIAN_POINT ( 'NONE',  ( 18.58859047265045561, -296.2481679979908904, -320.3485107564493433 ) ) ;
#7023=CARTESIAN_POINT ( 'NONE',  ( -60.02525093786476873, -289.5049175206884797, -343.9441087287246432 ) ) ;
#7024=CARTESIAN_POINT ( 'NONE',  ( 37.37463990632037536, -279.4841628664315749, -258.7612681658479801 ) ) ;
#7025=CARTESIAN_POINT ( 'NONE',  ( 15.43971002028817097, -292.6066879537513046, -214.2243466889837862 ) ) ;
#7027=CARTESIAN_POINT ( 'NONE',  ( -20.00487668688056075, -291.3390828561145440, -199.1550204795333912 ) ) ;
#7028=CARTESIAN_POINT ( 'NONE',  ( -37.70552466142714110, -293.0565156061199446, -345.3729781758001991 ) ) ;
#7031=CARTESIAN_POINT ( 'NONE',  ( -32.14665728274690792, -291.6270648105657983, -197.4718791760972181 ) ) ;
#7033=CARTESIAN_POINT ( 'NONE',  ( -21.33282851196157992, -271.7666405000204009, -200.3683826091710216 ) ) ;
#7034=CARTESIAN_POINT ( 'NONE',  ( -93.52545843255403213, -294.8955179977752437, -322.6892331384437398 ) ) ;
#7035=CARTESIAN_POINT ( 'NONE',  ( -111.3933866198906202, -285.6245445313695086, -289.6391917190264280 ) ) ;
#7036=CARTESIAN_POINT ( 'NONE',  ( -5.796726697909574177, -286.3120962107630021, -204.5148596655744768 ) ) ;
#7037=CARTESIAN_POINT ( 'NONE',  ( 33.91752932821798083, -277.3179731855609589, -289.1448868062686870 ) ) ;
#7038=CARTESIAN_POINT ( 'NONE',  ( -9.908448962836978069, -292.7122189930585137, -339.7820336625546815 ) ) ;
#7039=CARTESIAN_POINT ( 'NONE',  ( 13.06113443965657872, -296.0969690239382999, -324.6303517046920319 ) ) ;
#7040=CARTESIAN_POINT ( 'NONE',  ( 35.77521956815993320, -274.2557155123517987, -263.3982587461104004 ) ) ;
#7043=CARTESIAN_POINT ( 'NONE',  ( -103.0997286745691923, -295.6961550887062344, -310.3814374858926612 ) ) ;
#7044=CARTESIAN_POINT ( 'NONE',  ( 6.716206674132316756, -290.3683259345561396, -330.4271649894664620 ) ) ;
#7045=CARTESIAN_POINT ( 'NONE',  ( 201.2384769459594338, 294.9663689418843546, -54.00000000002624745 ) ) ;
#7046=CARTESIAN_POINT ( 'NONE',  ( -30.53256907643855911, -299.2151910733154523, -193.6690121210707218 ) ) ;
#7048=CARTESIAN_POINT ( 'NONE',  ( 34.09385243788444342, -287.9991247326987036, -254.8416302928420123 ) ) ;
#7050=CARTESIAN_POINT ( 'NONE',  ( -86.64440001091345778, -278.4452443927756917, -211.4525367236306295 ) ) ;
#7051=CARTESIAN_POINT ( 'NONE',  ( 30.81583674611254864, -294.6635482439505722, -305.9681812358531943 ) ) ;
#7052=CARTESIAN_POINT ( 'NONE',  ( -41.71335259280697727, -287.2462313559519202, -346.0127037148496925 ) ) ;
#7053=CARTESIAN_POINT ( 'NONE',  ( -44.78935280849671585, -295.4771217365113785, -347.0322411531286662 ) ) ;
#7054=CARTESIAN_POINT ( 'NONE',  ( 34.23637452811453841, -293.6949321124462813, -255.9158171768883392 ) ) ;
#7057=CARTESIAN_POINT ( 'NONE',  ( 37.87016018917535831, -288.9087604193013021, -257.4047721936249218 ) ) ;
#7058=CARTESIAN_POINT ( 'NONE',  ( -119.3990491898856732, -288.0523547857347353, -270.3284710469131937 ) ) ;
#7059=CARTESIAN_POINT ( 'NONE',  ( -62.00707101680345090, -279.0884357435809875, -197.4699962417320478 ) ) ;
#7060=CARTESIAN_POINT ( 'NONE',  ( -67.26996307630848548, -285.4456307076307553, -338.9631276106981659 ) ) ;
#7061=CARTESIAN_POINT ( 'NONE',  ( -111.7815602526666083, -283.3441965717582320, -253.1183362963863033 ) ) ;
#7062=CARTESIAN_POINT ( 'NONE',  ( 29.51046450980167180, -286.0669579147032096, -303.1040909402275361 ) ) ;
#7063=CARTESIAN_POINT ( 'NONE',  ( 26.61900499379244422, -277.9545973047178222, -311.0706754686984823 ) ) ;
#7064=CARTESIAN_POINT ( 'NONE',  ( -105.4374961801752875, -273.2392712410683657, -243.8578155381300689 ) ) ;
#7066=CARTESIAN_POINT ( 'NONE',  ( -108.7647745755792386, -278.3530741203107937, -285.4523219261550366 ) ) ;
#7067=CARTESIAN_POINT ( 'NONE',  ( -110.3823259807169421, -277.8613037742954361, -273.3543842450285979 ) ) ;
#7068=CARTESIAN_POINT ( 'NONE',  ( -18.63872135734161972, -275.3671001505113054, -195.9309720107538908 ) ) ;
#7069=CARTESIAN_POINT ( 'NONE',  ( -107.0513787054035078, -277.7565670481077973, -238.4754808204128267 ) ) ;
#7070=CARTESIAN_POINT ( 'NONE',  ( 82.92988855738929033, 83.04799596232011538, -299.9466387458070926 ) ) ;
#7071=CARTESIAN_POINT ( 'NONE',  ( -112.5622897402321740, -298.1467245017408345, -256.9272357375537013 ) ) ;
#7072=CARTESIAN_POINT ( 'NONE',  ( -85.28047601435908120, -280.1948066931273047, -330.5268031993605859 ) ) ;
#7074=CARTESIAN_POINT ( 'NONE',  ( -17.09966293588080077, -287.3992388870588570, -199.8489406817098200 ) ) ;
#7075=CARTESIAN_POINT ( 'NONE',  ( -1.468010098879991121, -288.2813009617613602, -203.3756540442568053 ) ) ;
#7076=CARTESIAN_POINT ( 'NONE',  ( 35.22440129381648433, -287.0171186732558795, -279.1959124088705266 ) ) ;
#7077=CARTESIAN_POINT ( 'NONE',  ( -93.87025930839122623, -284.7716884051310444, -218.0906233700659129 ) ) ;
#7078=CARTESIAN_POINT ( 'NONE',  ( -3.967757526706389815, -278.8997267243151441, -204.5244298472641731 ) ) ;
#7079=CARTESIAN_POINT ( 'NONE',  ( -38.67038157317211500, -287.8957673897451741, -196.1251131226379982 ) ) ;
#7080=CARTESIAN_POINT ( 'NONE',  ( -1.613138504112029858, -279.0147793021048983, -205.9082077491523251 ) ) ;
#7081=CARTESIAN_POINT ( 'NONE',  ( -74.24652513619511751, -278.8690315782885705, -333.9164275119168792 ) ) ;
#7082=CARTESIAN_POINT ( 'NONE',  ( 30.22934423381503777, -275.6707975466348444, -242.4408504447100370 ) ) ;
#7083=CARTESIAN_POINT ( 'NONE',  ( -7.090927681746135747, -287.4589500239404174, -340.7521223062466902 ) ) ;
#7085=CARTESIAN_POINT ( 'NONE',  ( -44.39418969742571619, -283.9419087698825592, -346.9285527955577209 ) ) ;
#7086=CARTESIAN_POINT ( 'NONE',  ( 22.47937911706563341, -282.6939875261372208, -318.7654306573768395 ) ) ;
#7090=CARTESIAN_POINT ( 'NONE',  ( -48.66068399534277233, -291.0550835054452818, -345.3287199756893529 ) ) ;
#7092=CARTESIAN_POINT ( 'NONE',  ( -107.9057941361184305, -289.6154458966639140, -240.7975101447190127 ) ) ;
#7093=CARTESIAN_POINT ( 'NONE',  ( -36.47075185634856354, -297.2604951136947875, -197.1997627011453176 ) ) ;
#7094=CARTESIAN_POINT ( 'NONE',  ( 38.25551345877767773, -293.0780124340349175, -284.5167600108106285 ) ) ;
#7095=CARTESIAN_POINT ( 'NONE',  ( -111.0305539148856582, -289.0214017338840335, -271.1738775337034326 ) ) ;
#7096=CARTESIAN_POINT ( 'NONE',  ( 34.42319523733951314, -292.0276786710265924, -288.4656425308204462 ) ) ;
#7097=CARTESIAN_POINT ( 'NONE',  ( -15.72010934889362233, -289.9713115370194032, -340.5543608675225187 ) ) ;
#7098=CARTESIAN_POINT ( 'NONE',  ( -4.829096099716510437, -294.9805209788416391, -202.7746430608542312 ) ) ;
#7099=CARTESIAN_POINT ( 'NONE',  ( -10.26108672732496530, -290.6988631617981014, -340.3013855461616117 ) ) ;
#7100=CARTESIAN_POINT ( 'NONE',  ( -76.19917938228769572, -289.5343665863347269, -205.9572992815773773 ) ) ;
#7101=CARTESIAN_POINT ( 'NONE',  ( -108.6286968551104337, -292.8552351796186599, -246.8927161664981327 ) ) ;
#7102=CARTESIAN_POINT ( 'NONE',  ( -110.6257822262946604, -285.4860212947751847, -270.9230285595351120 ) ) ;
#7103=CARTESIAN_POINT ( 'NONE',  ( -2.918675998981901554, -294.5060914746232470, -203.5254114378927852 ) ) ;
#7106=CARTESIAN_POINT ( 'NONE',  ( -68.19420706344247662, -275.6289073083696621, -201.5972668998938104 ) ) ;
#7107=CARTESIAN_POINT ( 'NONE',  ( 35.72668069995849294, -280.7978797817931991, -274.0507588419442300 ) ) ;
#7108=CARTESIAN_POINT ( 'NONE',  ( -20.97594140799273177, -280.8421099611669547, -343.6071924052199620 ) ) ;
#7109=CARTESIAN_POINT ( 'NONE',  ( -77.00765004450929041, -294.7661319212363082, -336.2316186421426210 ) ) ;
#7110=CARTESIAN_POINT ( 'NONE',  ( -0.01613631748763947812, -272.7959631242477485, -206.4340675467720700 ) ) ;
#7111=CARTESIAN_POINT ( 'NONE',  ( -108.9979491427641136, -276.8939667428833218, -250.1472208473432488 ) ) ;
#7112=CARTESIAN_POINT ( 'NONE',  ( -67.03383423311878175, -298.9697968567703583, -203.1192200960973082 ) ) ;
#7113=CARTESIAN_POINT ( 'NONE',  ( -32.70012028322606312, -272.6842735674172786, -194.0784015736182084 ) ) ;
#7115=CARTESIAN_POINT ( 'NONE',  ( 8.610147779436365667, -295.8339420924097567, -327.9053352202059273 ) ) ;
#7117=CARTESIAN_POINT ( 'NONE',  ( 12.47228721121615003, -295.1398145241167299, -324.0138475432739824 ) ) ;
#7119=CARTESIAN_POINT ( 'NONE',  ( 31.35486059148992410, -285.9765145794269188, -301.3319001026927140 ) ) ;
#7120=CARTESIAN_POINT ( 'NONE',  ( -107.4593678003782458, -296.8207896077103101, -250.0507098084899269 ) ) ;
#7121=CARTESIAN_POINT ( 'NONE',  ( -112.2191501870833292, -284.3269071426077517, -288.3715275247583918 ) ) ;
#7122=CARTESIAN_POINT ( 'NONE',  ( 30.11507937956458747, -286.7372079471851407, -233.1651006806397390 ) ) ;
#7123=CARTESIAN_POINT ( 'NONE',  ( -64.97632907408589631, -297.3912319468601595, -340.4801984846240543 ) ) ;
#7124=CARTESIAN_POINT ( 'NONE',  ( 26.42306370415410299, -291.0241908030313311, -231.0953168893059910 ) ) ;
#7125=CARTESIAN_POINT ( 'NONE',  ( -106.0266406357846165, -278.1946908041737743, -235.7964893375063866 ) ) ;
#7126=CARTESIAN_POINT ( 'NONE',  ( -69.85430415644619018, -283.1237833571632336, -202.7746430608542312 ) ) ;
#7128=CARTESIAN_POINT ( 'NONE',  ( 29.17625045938557449, -285.9304288892359978, -239.3370506595847758 ) ) ;
#7131=CARTESIAN_POINT ( 'NONE',  ( -109.6646779096919886, -297.9597641865797755, -285.1150300007515170 ) ) ;
#7132=CARTESIAN_POINT ( 'NONE',  ( 31.48278798456017569, -282.5469119903268620, -237.0461362092005118 ) ) ;
#7133=CARTESIAN_POINT ( 'NONE',  ( -108.7942807330012158, -294.2642801701703661, -294.2971896536288909 ) ) ;
#7134=CARTESIAN_POINT ( 'NONE',  ( 35.13978117179284055, -281.6721582681755649, -279.4582361891523874 ) ) ;
#7135=CARTESIAN_POINT ( 'NONE',  ( -79.47519025333227205, -295.7711118491522484, -334.8108582020454946 ) ) ;
#7136=CARTESIAN_POINT ( 'NONE',  ( -94.16042442217737118, -298.7314441443371607, -223.4123825899095266 ) ) ;
#7137=CARTESIAN_POINT ( 'NONE',  ( -112.2334996200438582, -280.5006066897011578, -274.3884017989200856 ) ) ;
#7138=CARTESIAN_POINT ( 'NONE',  ( -109.3757370138529836, -295.4362798152733944, -283.6407202090755391 ) ) ;
#7139=ORIENTED_EDGE ( 'NONE', *, *, #24867, .T. ) ;
#7141=CARTESIAN_POINT ( 'NONE',  ( -26.47904842952123872, -284.8932935787976817, -344.2637591965354318 ) ) ;
#7142=CARTESIAN_POINT ( 'NONE',  ( 35.77081079830085031, -285.2666405000204577, -287.0812184334320705 ) ) ;
#7143=CARTESIAN_POINT ( 'NONE',  ( 31.11108745493102390, -274.2988428703843056, -235.4558935581463004 ) ) ;
#7144=CARTESIAN_POINT ( 'NONE',  ( -38.89545100498257568, -291.8654403850818539, -197.3776550423595779 ) ) ;
#7145=CARTESIAN_POINT ( 'NONE',  ( 36.12186651307747809, -283.1563243192268260, -276.7925661319537198 ) ) ;
#7146=CARTESIAN_POINT ( 'NONE',  ( 10.19473273332901186, -277.9837410051501365, -326.8122292550070256 ) ) ;
#7147=CARTESIAN_POINT ( 'NONE',  ( -55.49168060666269042, -284.8820700471522400, -344.3680002438806582 ) ) ;
#7148=CARTESIAN_POINT ( 'NONE',  ( 16.10452853613887214, -281.0680866321639542, -320.7398045616621971 ) ) ;
#7149=CARTESIAN_POINT ( 'NONE',  ( -97.22357734207655255, -281.1699180712141128, -225.1827164605083169 ) ) ;
#7150=CARTESIAN_POINT ( 'NONE',  ( -95.08788239902190753, -273.4085100799261454, -219.4260766293930374 ) ) ;
#7151=CARTESIAN_POINT ( 'NONE',  ( 37.63539790685170061, -275.1655360718625616, -252.7699371046462886 ) ) ;
#7152=CARTESIAN_POINT ( 'NONE',  ( 34.69567685560257075, -295.2294235094186092, -251.6013067403051195 ) ) ;
#7156=CARTESIAN_POINT ( 'NONE',  ( -47.48995389434674763, -293.3194205098727707, -345.4431958992966543 ) ) ;
#7157=CARTESIAN_POINT ( 'NONE',  ( 15.49562604702088642, -274.3318680299166772, -219.8279375278595467 ) ) ;
#7158=CARTESIAN_POINT ( 'NONE',  ( -27.95376492520366796, -293.6892561052258657, -194.5809552263336002 ) ) ;
#7159=CARTESIAN_POINT ( 'NONE',  ( -106.6379572354042296, -280.6233781216988064, -303.7686719486574702 ) ) ;
#7160=CARTESIAN_POINT ( 'NONE',  ( -4.786900107585593034, -293.6765280656847494, -201.0199778420223424 ) ) ;
#7161=CARTESIAN_POINT ( 'NONE',  ( -4.977042499739167347, -290.6251904383378246, -337.8337596082291725 ) ) ;
#7162=CARTESIAN_POINT ( 'NONE',  ( -106.1172279546642869, -276.9385234058473202, -240.8661150861728117 ) ) ;
#7163=CARTESIAN_POINT ( 'NONE',  ( -3.185369503373105537, -278.5174666350597477, -336.5023250997544437 ) ) ;
#7164=CARTESIAN_POINT ( 'NONE',  ( 18.13778201089037623, -292.3284865894563040, -320.0123873693774499 ) ) ;
#7165=CARTESIAN_POINT ( 'NONE',  ( 16.33108357850814585, -282.6644319118433941, -216.8129312042700008 ) ) ;
#7166=CARTESIAN_POINT ( 'NONE',  ( -73.69702880635465192, -284.4777452976173890, -206.6871859149378565 ) ) ;
#7168=CARTESIAN_POINT ( 'NONE',  ( -94.30417223308484154, -283.5732186842045053, -316.0686921172443817 ) ) ;
#7169=CARTESIAN_POINT ( 'NONE',  ( 16.99435925800993985, -281.8838132093619038, -216.1656443505091545 ) ) ;
#7170=CARTESIAN_POINT ( 'NONE',  ( -99.47545859961090287, -282.7489472816398575, -315.2538570478912447 ) ) ;
#7171=CARTESIAN_POINT ( 'NONE',  ( -112.8320463949825694, -279.3177547684487081, -284.3626656460864410 ) ) ;
#7173=CARTESIAN_POINT ( 'NONE',  ( -20.26228589976311056, -278.3568506892581809, -344.7860498234580291 ) ) ;
#7174=CARTESIAN_POINT ( 'NONE',  ( -92.08974858914540107, -299.6948066931273047, -226.7417163044926838 ) ) ;
#7176=CARTESIAN_POINT ( 'NONE',  ( -103.6668617920756787, -275.0136687236110333, -235.5933444221973332 ) ) ;
#7177=CARTESIAN_POINT ( 'NONE',  ( -111.1215563367978376, -276.4260836690726819, -281.6915911053656032 ) ) ;
#7178=CARTESIAN_POINT ( 'NONE',  ( -67.94153441006896799, -293.4161115380208571, -200.7939066959690706 ) ) ;
#7179=CARTESIAN_POINT ( 'NONE',  ( 8.285327411402866105, -293.7575907092848979, -327.5406761253193508 ) ) ;
#7180=CARTESIAN_POINT ( 'NONE',  ( -36.09413305362367197, -288.5445924022116628, -347.3025643310726309 ) ) ;
#7182=CARTESIAN_POINT ( 'NONE',  ( 17.12867446459954124, -292.8689781493878854, -324.0235240223855158 ) ) ;
#7183=CARTESIAN_POINT ( 'NONE',  ( -97.21202249259219741, -283.5491817299816830, -227.1888439198559695 ) ) ;
#7184=CARTESIAN_POINT ( 'NONE',  ( -94.40425624975429741, -293.0751925236358488, -222.8572660269012999 ) ) ;
#7185=CARTESIAN_POINT ( 'NONE',  ( -22.29957616885191030, -284.7280169917509625, -198.1669211354738707 ) ) ;
#7186=CARTESIAN_POINT ( 'NONE',  ( 19.74563475441328819, -283.5179939348461176, -316.6657268384461759 ) ) ;
#7187=CARTESIAN_POINT ( 'NONE',  ( -78.00158110369487474, -290.5252851946589203, -335.5352868487544242 ) ) ;
#7188=CARTESIAN_POINT ( 'NONE',  ( -49.15803158862561162, -280.3898404293923932, -198.2614456371258314 ) ) ;
#7189=CARTESIAN_POINT ( 'NONE',  ( 23.70320921492129784, -292.9668288521231716, -316.6377618017401119 ) ) ;
#7190=CARTESIAN_POINT ( 'NONE',  ( -71.82482149821827022, -290.2991598961791624, -339.0275083183964853 ) ) ;
#7191=CARTESIAN_POINT ( 'NONE',  ( -107.6725686388678440, -290.6446161164286082, -301.6866124972198122 ) ) ;
#7192=CARTESIAN_POINT ( 'NONE',  ( -108.6653612838779139, -284.9247893153510063, -254.7484792412284094 ) ) ;
#7195=CARTESIAN_POINT ( 'NONE',  ( -16.81832942683857723, -296.6503936476161698, -343.3476081012445889 ) ) ;
#7196=CARTESIAN_POINT ( 'NONE',  ( -66.75045764000135762, -294.1142937034701959, -341.0040009966007233 ) ) ;
#7197=CARTESIAN_POINT ( 'NONE',  ( -104.6536365235664761, -277.9972614360513603, -241.5078397260232066 ) ) ;
#7198=CARTESIAN_POINT ( 'NONE',  ( -90.11608427741597893, -272.8379850721510138, -214.3027349565816166 ) ) ;
#7199=CARTESIAN_POINT ( 'NONE',  ( -94.49241062865399954, -294.3795063799121863, -316.9051871735808277 ) ) ;
#7200=CARTESIAN_POINT ( 'NONE',  ( 16.34818114384753329, -278.0365607360602667, -321.3058985051895320 ) ) ;
#7201=CARTESIAN_POINT ( 'NONE',  ( -110.3400107804503847, -270.8703530188331001, -256.5917214264551944 ) ) ;
#7202=CARTESIAN_POINT ( 'NONE',  ( 31.19371124689212493, -294.4082951049963413, -244.0927360039654275 ) ) ;
#7203=CARTESIAN_POINT ( 'NONE',  ( -18.12629589025442556, -295.8782519814267289, -341.1071024106926757 ) ) ;
#7205=CARTESIAN_POINT ( 'NONE',  ( -103.0138546998814775, -294.0651481195229167, -307.0352826579660928 ) ) ;
#7206=CARTESIAN_POINT ( 'NONE',  ( -3.474620760922319640, -299.1171511841361621, -193.4594115620958235 ) ) ;
#7207=CARTESIAN_POINT ( 'NONE',  ( -91.66225793563351942, -275.2782973076661506, -218.6289031468443227 ) ) ;
#7208=CARTESIAN_POINT ( 'NONE',  ( -73.65123802759283933, -290.4880025271413615, -333.9760928769686075 ) ) ;
#7210=CARTESIAN_POINT ( 'NONE',  ( -6.752185930356357169, -294.9724303683275934, -336.6662392629854708 ) ) ;
#7212=CARTESIAN_POINT ( 'NONE',  ( -104.7165239969798876, -280.9769677934530705, -236.4951618567751268 ) ) ;
#7213=CARTESIAN_POINT ( 'NONE',  ( -71.00243563160469762, -278.3020554667772899, -201.6570194123836472 ) ) ;
#7214=CARTESIAN_POINT ( 'NONE',  ( -50.08479655238178196, -282.5591333045410352, -346.2497843848386196 ) ) ;
#7215=CARTESIAN_POINT ( 'NONE',  ( 18.02198024882880034, -274.1683619831264878, -216.9163685676203386 ) ) ;
#7216=CARTESIAN_POINT ( 'NONE',  ( -97.92776169824443855, -277.5748366934224123, -224.1254826648542746 ) ) ;
#7217=CARTESIAN_POINT ( 'NONE',  ( 13.92988305839977414, -278.7687763035351054, -215.3240152272078660 ) ) ;
#7218=CARTESIAN_POINT ( 'NONE',  ( -37.80895721098180928, -296.7310026960128084, -196.8694507646536067 ) ) ;
#7219=CARTESIAN_POINT ( 'NONE',  ( 30.20466255269252542, -277.1216036762295403, -237.6473325055321197 ) ) ;
#7221=CARTESIAN_POINT ( 'NONE',  ( 3.276644636312318504, -290.6147296812558807, -206.8283415308592055 ) ) ;
#7222=CARTESIAN_POINT ( 'NONE',  ( -84.26634997801217253, -291.4270372459754981, -209.2441245203598896 ) ) ;
#7223=CARTESIAN_POINT ( 'NONE',  ( 35.84391337528088428, -277.3320258065396047, -253.1618620851873800 ) ) ;
#7224=CARTESIAN_POINT ( 'NONE',  ( -103.7909281743501708, -271.0139915186837811, -235.4708296132491512 ) ) ;
#7225=CARTESIAN_POINT ( 'NONE',  ( -114.1792412848347169, -283.7541924397377784, -269.9724163247458932 ) ) ;
#7227=CARTESIAN_POINT ( 'NONE',  ( -106.1944638811755226, -282.9424797285483351, -240.4950376771912204 ) ) ;
#7229=CARTESIAN_POINT ( 'NONE',  ( 21.32035684398580955, -291.7309960939639950, -226.2488342322953372 ) ) ;
#7230=CARTESIAN_POINT ( 'NONE',  ( -69.28533722039857423, -283.7669347865880809, -203.3361320070691534 ) ) ;
#7233=CARTESIAN_POINT ( 'NONE',  ( -53.60728416713134692, -293.2605465356435843, -343.6294976467989386 ) ) ;
#7234=CARTESIAN_POINT ( 'NONE',  ( -111.8523100230623157, -282.8243325068079344, -286.8194523056383787 ) ) ;
#7235=CARTESIAN_POINT ( 'NONE',  ( -110.2796499548566800, -280.0055263922336053, -281.6081571790532507 ) ) ;
#7236=CARTESIAN_POINT ( 'NONE',  ( -113.5074147319497513, -285.6544849095171230, -278.5337942202795034 ) ) ;
#7237=CARTESIAN_POINT ( 'NONE',  ( 4.725366358314717630, -286.6376670810212204, -210.6388719559611218 ) ) ;
#7238=CARTESIAN_POINT ( 'NONE',  ( -97.35579628699115062, -279.3872387993422990, -312.9703550283261393 ) ) ;
#7239=CARTESIAN_POINT ( 'NONE',  ( -107.2679349521096981, -279.0686007766782382, -292.0463360408438689 ) ) ;
#7240=CARTESIAN_POINT ( 'NONE',  ( -77.66408300951567867, -287.4935398090840977, -206.7017727117505217 ) ) ;
#7241=EDGE_LOOP ( 'NONE', ( #74576, #14622 ) ) ;
#7242=CARTESIAN_POINT ( 'NONE',  ( -29.05750026640263783, -297.9865096745180608, -193.3613442771316784 ) ) ;
#7243=CARTESIAN_POINT ( 'NONE',  ( -48.27759395506573981, -291.1717583829959040, -344.2526611745329319 ) ) ;
#7245=CARTESIAN_POINT ( 'NONE',  ( -88.47809603358389552, -280.1948066931273615, -334.5364918783848793 ) ) ;
#7247=CARTESIAN_POINT ( 'NONE',  ( 37.56701494694144117, -292.1294505906153631, -284.4002304093277758 ) ) ;
#7248=CARTESIAN_POINT ( 'NONE',  ( 2.808707373818427389, -288.1218635581265630, -208.5658711673335688 ) ) ;
#7249=CARTESIAN_POINT ( 'NONE',  ( -24.72539527704555340, -281.9754725635006594, -197.4309948290255363 ) ) ;
#7250=CARTESIAN_POINT ( 'NONE',  ( 15.87570614894008614, -288.2137928377180174, -215.5294304189747834 ) ) ;
#7251=CARTESIAN_POINT ( 'NONE',  ( -23.38535074789511370, -290.1926157370633632, -345.6380130623340960 ) ) ;
#7252=CARTESIAN_POINT ( 'NONE',  ( -64.76353949753462302, -285.4104154463406076, -340.1683051118224057 ) ) ;
#7253=CARTESIAN_POINT ( 'NONE',  ( -113.2368464688460818, -278.8813791914287776, -257.3639349635557778 ) ) ;
#7255=CARTESIAN_POINT ( 'NONE',  ( 21.15598079295905265, -292.2864592625681439, -318.2075177388838370 ) ) ;
#7256=CARTESIAN_POINT ( 'NONE',  ( 33.56509868952359454, -281.7690813911262353, -300.5176987633950034 ) ) ;
#7257=CARTESIAN_POINT ( 'NONE',  ( -77.24785468263895893, -275.3712703558093153, -207.7642785429671619 ) ) ;
#7258=CARTESIAN_POINT ( 'NONE',  ( 10.64812456238590066, -296.9090924074130271, -330.4860931364851808 ) ) ;
#7259=CARTESIAN_POINT ( 'NONE',  ( 0.7076817878556337371, -272.7920367444243084, -204.5720357498089186 ) ) ;
#7261=CARTESIAN_POINT ( 'NONE',  ( -94.83539817078383294, -278.6951295816203356, -225.2581365094856949 ) ) ;
#7262=CARTESIAN_POINT ( 'NONE',  ( 36.89660199557103226, -276.5196711305298436, -251.4750591648150930 ) ) ;
#7263=CARTESIAN_POINT ( 'NONE',  ( -110.8354741793802276, -273.9030467697824065, -267.6355640499449464 ) ) ;
#7264=CARTESIAN_POINT ( 'NONE',  ( -95.16541780068362755, -282.9259802854631403, -320.8510960763929347 ) ) ;
#7265=CARTESIAN_POINT ( 'NONE',  ( -80.13461248654070346, -293.2245296477840384, -209.9100366727946323 ) ) ;
#7266=CARTESIAN_POINT ( 'NONE',  ( -96.32987636094588879, -274.8068644004699195, -222.1034674048001420 ) ) ;
#7267=CARTESIAN_POINT ( 'NONE',  ( -62.72800018497400032, -298.9339808649056067, -198.0870252002743257 ) ) ;
#7268=CARTESIAN_POINT ( 'NONE',  ( 36.51944549281796526, -295.3965629740329177, -258.2578604923841112 ) ) ;
#7269=CARTESIAN_POINT ( 'NONE',  ( -69.82750888952243429, -281.4807601740003520, -337.7896654513637031 ) ) ;
#7270=CARTESIAN_POINT ( 'NONE',  ( -74.66492877972062558, -291.2360943320602473, -203.0356332492932552 ) ) ;
#7271=CARTESIAN_POINT ( 'NONE',  ( -40.82706062568297511, -272.0283339704262744, -195.7469068541524280 ) ) ;
#7272=CARTESIAN_POINT ( 'NONE',  ( -54.80130261255236945, -287.4314623565190914, -196.1883285346809771 ) ) ;
#7273=CARTESIAN_POINT ( 'NONE',  ( -95.35059346602918140, -290.1009269421457475, -225.5370801424006686 ) ) ;
#7275=CARTESIAN_POINT ( 'NONE',  ( -111.9935966042498308, -288.9214562681422649, -286.6614446004053320 ) ) ;
#7276=CARTESIAN_POINT ( 'NONE',  ( -73.55913816900171298, -289.2136750876487099, -333.7820373800358880 ) ) ;
#7278=CARTESIAN_POINT ( 'NONE',  ( -65.77558574881582842, -286.7685004050736666, -199.1219766837695602 ) ) ;
#7279=CARTESIAN_POINT ( 'NONE',  ( -94.46692208612743968, -278.2430617321524551, -315.8651140816054976 ) ) ;
#7280=CARTESIAN_POINT ( 'NONE',  ( 21.08392122010786096, -291.7998335950834417, -220.6626927068153634 ) ) ;
#7281=CARTESIAN_POINT ( 'NONE',  ( -113.4972347800642041, -285.0653552029529010, -281.3974856930398118 ) ) ;
#7282=CARTESIAN_POINT ( 'NONE',  ( -113.1153965253515565, -284.7120382297592869, -284.2217233150922198 ) ) ;
#7283=CARTESIAN_POINT ( 'NONE',  ( 13.34672591524345009, -281.1181539504035527, -217.7285905783485020 ) ) ;
#7284=CARTESIAN_POINT ( 'NONE',  ( 194.3816077206797672, 279.0927965383107221, -125.9308262313876554 ) ) ;
#7285=CARTESIAN_POINT ( 'NONE',  ( 83.43343483694488327, 83.57203687522600433, -301.5415206557701140 ) ) ;
#7286=CARTESIAN_POINT ( 'NONE',  ( -22.83531149767027557, -108.3062553589070376, -359.1681096793552115 ) ) ;
#7287=CARTESIAN_POINT ( 'NONE',  ( -91.23458003854895537, -272.4580642510734947, -220.8636993540350488 ) ) ;
#7288=CARTESIAN_POINT ( 'NONE',  ( 17.52601395158817610, -273.7800237770179592, -221.6673662946266461 ) ) ;
#7289=CARTESIAN_POINT ( 'NONE',  ( -2.001332507245941361, -294.1044473235040755, -338.7027986749537263 ) ) ;
#7290=CARTESIAN_POINT ( 'NONE',  ( -97.10692441846769896, -247.3327781681390434, -331.7524723150551722 ) ) ;
#7291=CARTESIAN_POINT ( 'NONE',  ( -5.305412031941359352, -273.1498058260812627, -200.8846865860590754 ) ) ;
#7292=CARTESIAN_POINT ( 'NONE',  ( -39.22298429835362299, -299.8887444167067429, -196.1371374432262087 ) ) ;
#7293=CARTESIAN_POINT ( 'NONE',  ( 36.14846292514583581, -288.8760192597929404, -271.0239987986652750 ) ) ;
#7295=CARTESIAN_POINT ( 'NONE',  ( 22.11203495250237694, -295.1474022478846564, -318.9417577962707355 ) ) ;
#7296=CARTESIAN_POINT ( 'NONE',  ( -22.45341665638626338, -286.7401623425297430, -198.7806865494790145 ) ) ;
#7297=CARTESIAN_POINT ( 'NONE',  ( -35.51730267654592410, -272.9948440623159627, -193.6788546413600045 ) ) ;
#7298=CARTESIAN_POINT ( 'NONE',  ( 38.69058855379418560, -294.2113767598840468, -258.9026380222433659 ) ) ;
#7299=CARTESIAN_POINT ( 'NONE',  ( 8.874196962227477670, -294.9294089835647128, -331.8722369708993938 ) ) ;
#7300=CARTESIAN_POINT ( 'NONE',  ( -110.2457897413033692, -290.7798233996524004, -265.7377335876513484 ) ) ;
#7301=ORIENTED_EDGE ( 'NONE', *, *, #86873, .T. ) ;
#7302=CARTESIAN_POINT ( 'NONE',  ( -87.10669878723285819, -275.2859343075214724, -213.4341772667394537 ) ) ;
#7303=CARTESIAN_POINT ( 'NONE',  ( 32.19907589617695720, -273.9325119451387422, -238.1086016015925679 ) ) ;
#7305=CARTESIAN_POINT ( 'NONE',  ( -108.6017983359425330, -277.6910922696535522, -299.3701735770973755 ) ) ;
#7306=AXIS2_PLACEMENT_3D ( 'NONE', #49041, #62320, #91160 ) ;
#7307=CARTESIAN_POINT ( 'NONE',  ( -4.938610846734867721, -272.8859581490106052, -204.0411808673291034 ) ) ;
#7308=CARTESIAN_POINT ( 'NONE',  ( -81.26716764257807313, -274.5190730836419561, -211.6051682571911954 ) ) ;
#7309=CARTESIAN_POINT ( 'NONE',  ( 34.94136667986096256, -276.6522269190517136, -282.4392749586534137 ) ) ;
#7310=CARTESIAN_POINT ( 'NONE',  ( 31.62381642964157891, -276.8972517539813794, -238.3339914456489907 ) ) ;
#7311=CARTESIAN_POINT ( 'NONE',  ( 0.2051289676536661166, -274.5753082265285911, -335.7551433604197655 ) ) ;
#7312=CARTESIAN_POINT ( 'NONE',  ( -107.6986632188032473, -296.9416090447183478, -290.2052711020807010 ) ) ;
#7313=CARTESIAN_POINT ( 'NONE',  ( -0.4783833154159193857, -293.1269915589218726, -334.1096994262956628 ) ) ;
#7315=CARTESIAN_POINT ( 'NONE',  ( -108.5970784161944920, -278.6756281051976885, -299.3817652547846819 ) ) ;
#7316=EDGE_CURVE ( 'NONE', #66639, #69774, #58267, .T. ) ;
#7317=CARTESIAN_POINT ( 'NONE',  ( -43.20497315338152333, -277.2949324147015204, -343.1252714782054909 ) ) ;
#7318=CARTESIAN_POINT ( 'NONE',  ( 38.07360725524704037, -286.0739223711511841, -257.4064627545597546 ) ) ;
#7319=CARTESIAN_POINT ( 'NONE',  ( -87.36587989630380946, -297.7475330820072941, -326.5344579262251727 ) ) ;
#7321=CARTESIAN_POINT ( 'NONE',  ( 35.43606684423092190, -286.6508172190175401, -262.8779127012985555 ) ) ;
#7322=CARTESIAN_POINT ( 'NONE',  ( -68.48392182479585699, -275.7068954339067091, -337.5177131985232677 ) ) ;
#7323=CARTESIAN_POINT ( 'NONE',  ( -85.50448027146268259, -276.3079747631875307, -326.0678421554713395 ) ) ;
#7324=CARTESIAN_POINT ( 'NONE',  ( -6.981474314252575475, -284.6539601972892797, -338.9551571135510244 ) ) ;
#7325=CARTESIAN_POINT ( 'NONE',  ( 7.836818112054698027, -277.6246654281800943, -328.2707868051127775 ) ) ;
#7326=CARTESIAN_POINT ( 'NONE',  ( 37.70778159425776721, -273.7843746852797722, -257.0949468214871558 ) ) ;
#7327=CARTESIAN_POINT ( 'NONE',  ( 23.13199988185597888, -275.6329188942714836, -229.2677022577485104 ) ) ;
#7328=CARTESIAN_POINT ( 'NONE',  ( -83.46261069444261693, -281.4221282114945097, -210.9412948250862314 ) ) ;
#7330=CARTESIAN_POINT ( 'NONE',  ( 35.01367428307751339, -289.7512843928762436, -292.1779677071431820 ) ) ;
#7331=CARTESIAN_POINT ( 'NONE',  ( 35.48612735234511462, -291.3212389420839941, -252.3888785349612931 ) ) ;
#7333=CARTESIAN_POINT ( 'NONE',  ( -39.16288030708625456, -296.8237485672630100, -196.9741648151990887 ) ) ;
#7334=CARTESIAN_POINT ( 'NONE',  ( -86.73348826152849256, -289.4967310613776590, -214.8724866495738013 ) ) ;
#7335=CARTESIAN_POINT ( 'NONE',  ( -102.0362518552990423, -259.7623939308359695, -328.6249738900723969 ) ) ;
#7337=CARTESIAN_POINT ( 'NONE',  ( -108.1622392593899349, -288.6682118485084629, -298.7716615952896291 ) ) ;
#7338=CARTESIAN_POINT ( 'NONE',  ( -46.36266841555873697, -284.1790391573577494, -194.9118227992420032 ) ) ;
#7339=CARTESIAN_POINT ( 'NONE',  ( -5.763761739604193579, -284.0539317238017247, -336.8445880951425693 ) ) ;
#7340=CARTESIAN_POINT ( 'NONE',  ( -95.23796663636437643, -284.7263841119616359, -315.1099008191312123 ) ) ;
#7341=CARTESIAN_POINT ( 'NONE',  ( -111.3152682984157451, -292.7164615455351964, -255.9300100085924328 ) ) ;
#7342=CARTESIAN_POINT ( 'NONE',  ( -7.702645710841940385, -274.7632777462546301, -199.2603914410591699 ) ) ;
#7343=CARTESIAN_POINT ( 'NONE',  ( -86.46713220710074665, -287.8076055874947201, -327.8407148384625316 ) ) ;
#7344=CARTESIAN_POINT ( 'NONE',  ( -80.22618522096833260, -277.6151522787772592, -334.3777930783103329 ) ) ;
#7345=CARTESIAN_POINT ( 'NONE',  ( 34.33651968054503101, -295.8020994586047436, -291.2416911104346582 ) ) ;
#7347=CARTESIAN_POINT ( 'NONE',  ( -54.49178911615187815, -294.3376638359846424, -195.3683826091709363 ) ) ;
#7348=CARTESIAN_POINT ( 'NONE',  ( -76.40332558018849340, -282.2709157401953917, -332.6742866197554918 ) ) ;
#7349=CARTESIAN_POINT ( 'NONE',  ( -101.6823991907854463, -277.0691194793241152, -231.7209270219530595 ) ) ;
#7350=CARTESIAN_POINT ( 'NONE',  ( -29.14603860014715764, -296.5530167252624665, -194.1633003519424676 ) ) ;
#7351=CARTESIAN_POINT ( 'NONE',  ( 5.449747793456863221, -275.8044679810632260, -329.6923719141394145 ) ) ;
#7352=CARTESIAN_POINT ( 'NONE',  ( -66.85939642382594172, -293.1782835180126767, -202.8376897577792306 ) ) ;
#7353=CARTESIAN_POINT ( 'NONE',  ( 35.85612424714413748, -294.4626086341283440, -268.0186931386346600 ) ) ;
#7354=CARTESIAN_POINT ( 'NONE',  ( -19.54178905977980918, -293.7018708416291588, -195.9981090741242724 ) ) ;
#7355=CARTESIAN_POINT ( 'NONE',  ( 37.87552115377394557, -295.0442818344714055, -284.4201210769314798 ) ) ;
#7356=CARTESIAN_POINT ( 'NONE',  ( -75.65986327579751958, -295.4119945539263767, -332.5547311101244645 ) ) ;
#7357=CARTESIAN_POINT ( 'NONE',  ( -95.64335279893977315, -291.9027365869796427, -317.5407528813690874 ) ) ;
#7358=CARTESIAN_POINT ( 'NONE',  ( -65.25020913368327058, -283.5736460396396410, -342.1396242093028377 ) ) ;
#7359=CARTESIAN_POINT ( 'NONE',  ( -57.76549615179668962, -271.9308735383560816, -197.3465018183667610 ) ) ;
#7360=CARTESIAN_POINT ( 'NONE',  ( 38.97555232233433031, -287.2575177201455290, -260.1299409768067790 ) ) ;
#7361=CARTESIAN_POINT ( 'NONE',  ( -72.40499749212899872, -279.4983972245187829, -336.2725132946476378 ) ) ;
#7362=CARTESIAN_POINT ( 'NONE',  ( -94.29749217648718229, -284.2601039909745850, -224.3038033710650723 ) ) ;
#7364=CARTESIAN_POINT ( 'NONE',  ( 2.105958780920293094, -286.5242751722619801, -334.2098248602603121 ) ) ;
#7365=CARTESIAN_POINT ( 'NONE',  ( -47.92246533766702044, -278.0586734568408360, -195.2857899559915325 ) ) ;
#7366=CARTESIAN_POINT ( 'NONE',  ( 138.4517698930976621, 181.0451598467585939, -241.7086681466011271 ) ) ;
#7367=CARTESIAN_POINT ( 'NONE',  ( -106.2338551108908717, -283.7345201533813110, -294.8399708850815273 ) ) ;
#7368=CARTESIAN_POINT ( 'NONE',  ( 20.75488144871690466, -282.0795940391786871, -220.4132701381974186 ) ) ;
#7369=CARTESIAN_POINT ( 'NONE',  ( -85.02792095063060174, -288.7504108396719289, -330.5857798872023636 ) ) ;
#7370=CARTESIAN_POINT ( 'NONE',  ( -106.6995022861665063, -280.5613197533720040, -238.6755537127948230 ) ) ;
#7371=CARTESIAN_POINT ( 'NONE',  ( -113.5542500113674294, -279.9590010970384810, -263.0776403166724435 ) ) ;
#7372=CARTESIAN_POINT ( 'NONE',  ( -6.767482008568397767, -280.2983314334559282, -204.0585803137349785 ) ) ;
#7373=CARTESIAN_POINT ( 'NONE',  ( -33.99153014528766903, -276.0743977868228285, -195.7915319182122289 ) ) ;
#7374=CARTESIAN_POINT ( 'NONE',  ( 38.81654538241593144, -293.6941541911065201, -281.7154845770832026 ) ) ;
#7375=CARTESIAN_POINT ( 'NONE',  ( -0.1943082086063979974, -286.5759808413779410, -335.1656272501982698 ) ) ;
#7376=CARTESIAN_POINT ( 'NONE',  ( -61.45494562234897984, -293.3443279717359360, -198.0214343523827552 ) ) ;
#7377=CARTESIAN_POINT ( 'NONE',  ( -109.1904178402274397, -295.2803978796736146, -284.9834920409502956 ) ) ;
#7378=CARTESIAN_POINT ( 'NONE',  ( -6.637615445609045040, -284.5660254688896771, -338.1878864456475640 ) ) ;
#7379=CARTESIAN_POINT ( 'NONE',  ( -107.9911126678050550, -295.9746349995157289, -288.8699270060547519 ) ) ;
#7380=ADVANCED_FACE ( 'NONE', ( #489 ), #76310, .T. ) ;
#7381=CARTESIAN_POINT ( 'NONE',  ( -112.2604165958704954, -291.4259945195586852, -286.7525314066531905 ) ) ;
#7382=CARTESIAN_POINT ( 'NONE',  ( 34.33226316028071068, -282.3938069907771364, -284.8024528873946224 ) ) ;
#7383=CARTESIAN_POINT ( 'NONE',  ( -111.5876062096892696, -271.8581163455078809, -250.6548316373763896 ) ) ;
#7384=CARTESIAN_POINT ( 'NONE',  ( -96.30754671483715867, -290.5381907459117201, -319.7408516773059546 ) ) ;
#7385=CARTESIAN_POINT ( 'NONE',  ( -71.20821920759951240, -281.6340472725624977, -338.1354816430568917 ) ) ;
#7386=CARTESIAN_POINT ( 'NONE',  ( -113.1117357226714972, -290.7145117023840157, -284.0240004984877373 ) ) ;
#7387=CARTESIAN_POINT ( 'NONE',  ( 4.734086419195035589, -286.9708946122954671, -210.6191333610420884 ) ) ;
#7389=CARTESIAN_POINT ( 'NONE',  ( -100.4238177162668393, -246.2515245119496115, -332.5401888311394032 ) ) ;
#7390=CARTESIAN_POINT ( 'NONE',  ( -111.1600279138487934, -270.9246594666713008, -270.3403961019906774 ) ) ;
#7391=CARTESIAN_POINT ( 'NONE',  ( -102.2945453730720970, -278.2075512087710081, -236.5799876957273966 ) ) ;
#7392=CARTESIAN_POINT ( 'NONE',  ( -39.69744901629324119, -278.9422343666826123, -197.0772920184110149 ) ) ;
#7393=CARTESIAN_POINT ( 'NONE',  ( 36.56675697029471905, -274.9467652579022001, -248.6507670799472578 ) ) ;
#7394=CARTESIAN_POINT ( 'NONE',  ( 181.3594537276159713, 251.3396015629845692, -165.1358875192213134 ) ) ;
#7395=CARTESIAN_POINT ( 'NONE',  ( -39.55188914467541395, -278.5996758072924990, -193.9693651698094072 ) ) ;
#7396=CARTESIAN_POINT ( 'NONE',  ( -91.96183380851151412, -281.8567976975985516, -321.2383014722413463 ) ) ;
#7397=CARTESIAN_POINT ( 'NONE',  ( -84.60389220254988629, -299.1712945176369089, -210.8610405742479372 ) ) ;
#7399=CARTESIAN_POINT ( 'NONE',  ( -105.7704830759360135, -291.3874835410810533, -244.6149867537183411 ) ) ;
#7400=CARTESIAN_POINT ( 'NONE',  ( 22.35253574138633326, -286.8322729737879513, -313.2311737645909488 ) ) ;
#7401=CARTESIAN_POINT ( 'NONE',  ( -38.36438704365086494, -274.6910569366528421, -193.4698512576767087 ) ) ;
#7402=CARTESIAN_POINT ( 'NONE',  ( -93.77838007488207950, -273.2082476322101456, -224.0392921260430796 ) ) ;
#7406=CARTESIAN_POINT ( 'NONE',  ( -107.1909812488175646, -280.8455200767294286, -241.5445928190535767 ) ) ;
#7408=CARTESIAN_POINT ( 'NONE',  ( -5.436336988437288298, -281.5617868795328604, -204.3590431843336717 ) ) ;
#7409=CARTESIAN_POINT ( 'NONE',  ( 22.92967474464701993, -282.6865176902531971, -224.0653042454112835 ) ) ;
#7410=CARTESIAN_POINT ( 'NONE',  ( -109.1573545956944713, -283.7995885584018652, -256.0111973508373353 ) ) ;
#7411=CARTESIAN_POINT ( 'NONE',  ( -71.53128412206604025, -281.4560224062233260, -204.4534078623156859 ) ) ;
#7412=CARTESIAN_POINT ( 'NONE',  ( -93.42900568078000845, -271.7057625159539498, -222.5407886399894721 ) ) ;
#7414=CARTESIAN_POINT ( 'NONE',  ( 30.40553344078523068, -276.8258151589418503, -306.7291272325348928 ) ) ;
#7416=CARTESIAN_POINT ( 'NONE',  ( 35.65144221479864228, -277.7742414586551831, -287.6502583164456723 ) ) ;
#7417=CARTESIAN_POINT ( 'NONE',  ( -59.51152465938343994, -275.9084964070916612, -343.4850208587597535 ) ) ;
#7420=CARTESIAN_POINT ( 'NONE',  ( -111.5133652729610390, -286.3583831934366231, -283.9501325348069258 ) ) ;
#7421=CARTESIAN_POINT ( 'NONE',  ( 35.45708788859575833, -292.6470921678688342, -262.5949118206045227 ) ) ;
#7422=EDGE_CURVE ( 'NONE', #37641, #11917, #68744, .T. ) ;
#7423=CARTESIAN_POINT ( 'NONE',  ( 39.47629699141587878, -286.8440308249012105, -265.8326795976899461 ) ) ;
#7424=CARTESIAN_POINT ( 'NONE',  ( -108.3706339366843707, -282.5199907487194082, -291.2118141177707002 ) ) ;
#7425=CARTESIAN_POINT ( 'NONE',  ( -70.49652195816902633, -282.0728041394958154, -336.0724916501939674 ) ) ;
#7426=CARTESIAN_POINT ( 'NONE',  ( 14.15300692814562922, -284.8615251816797240, -216.5348918934058418 ) ) ;
#7428=CARTESIAN_POINT ( 'NONE',  ( -2.225260288398726694, -283.7815079380501970, -334.8267560375776384 ) ) ;
#7429=CARTESIAN_POINT ( 'NONE',  ( 12.65082333798339675, -272.7485685126762291, -214.3833030623713398 ) ) ;
#7430=CARTESIAN_POINT ( 'NONE',  ( -97.42632129310945288, -282.3193136978437110, -317.2255897905537267 ) ) ;
#7431=CARTESIAN_POINT ( 'NONE',  ( -47.33909678044954461, -297.1793749872496733, -344.6918162647891677 ) ) ;
#7432=CARTESIAN_POINT ( 'NONE',  ( -97.85283191370568545, -283.1599014465709843, -225.6836823457252592 ) ) ;
#7433=CARTESIAN_POINT ( 'NONE',  ( -96.27524051113842063, -278.8857423555685386, -313.8590963136624055 ) ) ;
#7434=CARTESIAN_POINT ( 'NONE',  ( 36.04082636296087827, -289.7616302308222771, -286.6998084993668385 ) ) ;
#7437=CARTESIAN_POINT ( 'NONE',  ( 34.13241908337529651, -295.7889322477259952, -295.0321057524276966 ) ) ;
#7438=CARTESIAN_POINT ( 'NONE',  ( -54.43381538617030913, -275.2714312219372346, -343.4411264895401246 ) ) ;
#7439=CARTESIAN_POINT ( 'NONE',  ( -113.0112184758847320, -289.9166622764174690, -257.0088592312889659 ) ) ;
#7440=CARTESIAN_POINT ( 'NONE',  ( -12.76078324710743672, -293.1272320691778077, -340.0010074388002863 ) ) ;
#7441=CARTESIAN_POINT ( 'NONE',  ( -48.70047374889004033, -275.8844992550568804, -343.0229221647573468 ) ) ;
#7442=CARTESIAN_POINT ( 'NONE',  ( -68.54548304247643387, -295.7773204443063264, -202.9885613389541277 ) ) ;
#7443=CARTESIAN_POINT ( 'NONE',  ( -65.53150343221980734, -292.9908656688523934, -202.4757313526060045 ) ) ;
#7444=CARTESIAN_POINT ( 'NONE',  ( -114.2704648735229114, -281.0519495502701943, -270.3937649182068981 ) ) ;
#7445=CARTESIAN_POINT ( 'NONE',  ( 22.61477395183548467, -292.6692338763337489, -317.5830181715749632 ) ) ;
#7446=CARTESIAN_POINT ( 'NONE',  ( -98.76533831848146860, -291.5902516473811943, -311.2934915457029774 ) ) ;
#7447=CARTESIAN_POINT ( 'NONE',  ( -74.16790956180355465, -289.8094647211008805, -203.8945526027512472 ) ) ;
#7448=CARTESIAN_POINT ( 'NONE',  ( 27.55861952962299100, -289.4477770440237805, -305.1585738415649871 ) ) ;
#7450=CARTESIAN_POINT ( 'NONE',  ( -109.7813925020787593, -291.2188711344051057, -280.7023806571189652 ) ) ;
#7452=CARTESIAN_POINT ( 'NONE',  ( -40.30793926865678856, -290.2937017117659479, -346.9196100134480503 ) ) ;
#7453=CARTESIAN_POINT ( 'NONE',  ( -64.13344471534428237, -277.7246182546919613, -199.8745057071383826 ) ) ;
#7454=CARTESIAN_POINT ( 'NONE',  ( -35.34083299532585443, -280.4098703869225915, -193.3951366930848792 ) ) ;
#7455=CARTESIAN_POINT ( 'NONE',  ( 39.25662076447748206, -281.3209443646743466, -278.5205064152426644 ) ) ;
#7456=CARTESIAN_POINT ( 'NONE',  ( 37.44411412497085223, -285.6330496409593138, -276.6743678429252782 ) ) ;
#7458=CARTESIAN_POINT ( 'NONE',  ( 22.79893944653491644, -280.2907011003915159, -313.9026273621292944 ) ) ;
#7459=CARTESIAN_POINT ( 'NONE',  ( -26.87436509219875802, -284.1849662811917483, -196.0430288327169137 ) ) ;
#7460=CARTESIAN_POINT ( 'NONE',  ( -30.24964759220584298, -125.8449128503669527, -361.7634443971322753 ) ) ;
#7461=CARTESIAN_POINT ( 'NONE',  ( -108.9487845264195585, -277.3700243759020054, -243.8432954897286891 ) ) ;
#7462=CARTESIAN_POINT ( 'NONE',  ( -95.57280689031875909, -284.1493092877096842, -220.3752646503569110 ) ) ;
#7463=CARTESIAN_POINT ( 'NONE',  ( -47.31662083503962890, -298.8636883046322055, -197.7569371551957147 ) ) ;
#7464=CARTESIAN_POINT ( 'NONE',  ( -60.52944703691477457, -293.3466080621436163, -200.2448844830101393 ) ) ;
#7465=CARTESIAN_POINT ( 'NONE',  ( -105.0949417310843330, -274.4379548514282305, -234.9181851586274377 ) ) ;
#7466=CARTESIAN_POINT ( 'NONE',  ( 19.19526936679832119, -275.8732280863191022, -316.5940060058034078 ) ) ;
#7467=CARTESIAN_POINT ( 'NONE',  ( -83.57316182170224295, -297.6859669656770961, -329.4836663018785430 ) ) ;
#7468=CARTESIAN_POINT ( 'NONE',  ( -85.16301476901415413, -289.8581645878473978, -330.7791399507503911 ) ) ;
#7469=CARTESIAN_POINT ( 'NONE',  ( 19.98977024346277531, -278.9548693950283678, -221.1233832260824670 ) ) ;
#7470=CARTESIAN_POINT ( 'NONE',  ( -68.32681738763457702, -291.4896017467254978, -199.8561667211738211 ) ) ;
#7471=CARTESIAN_POINT ( 'NONE',  ( -65.40607646833963429, -290.7348041068386806, -202.7029073236534202 ) ) ;
#7472=CARTESIAN_POINT ( 'NONE',  ( -14.41819649820433646, -292.7547783979167093, -341.7719969028601668 ) ) ;
#7475=CARTESIAN_POINT ( 'NONE',  ( -107.4525815674616354, -290.3320298012379794, -249.7630531818940653 ) ) ;
#7477=CARTESIAN_POINT ( 'NONE',  ( -83.14512187467356341, -286.3836548251858858, -208.6923339555095254 ) ) ;
#7478=CARTESIAN_POINT ( 'NONE',  ( 26.47324843497312585, -301.4082689599840705, -200.3320873922942553 ) ) ;
#7479=CARTESIAN_POINT ( 'NONE',  ( -47.61199230273555116, -294.2384363786133008, -346.4356952810940129 ) ) ;
#7480=CARTESIAN_POINT ( 'NONE',  ( -113.6612436882926005, -285.9435643748756775, -264.3040664952717975 ) ) ;
#7481=CARTESIAN_POINT ( 'NONE',  ( -109.9941950075484414, -284.4859016005613626, -262.7479411179006092 ) ) ;
#7482=CARTESIAN_POINT ( 'NONE',  ( 28.47188256612149004, -276.6265065085495394, -237.2057250053155428 ) ) ;
#7483=CARTESIAN_POINT ( 'NONE',  ( 2.425238653974422842, -292.5369014915720527, -333.5922310729378069 ) ) ;
#7484=CARTESIAN_POINT ( 'NONE',  ( 6.683448190523597177, -296.2047645162321601, -329.9208869976035317 ) ) ;
#7485=CARTESIAN_POINT ( 'NONE',  ( -16.28153566092877469, -275.5688269709810925, -340.7251504719338868 ) ) ;
#7488=CARTESIAN_POINT ( 'NONE',  ( -64.26276884511517551, -295.0607372581387722, -342.4790793419596184 ) ) ;
#7489=CARTESIAN_POINT ( 'NONE',  ( 18.92982692873014017, -290.1539974459580549, -319.1705488075295989 ) ) ;
#7490=CARTESIAN_POINT ( 'NONE',  ( -40.51493896710162090, -296.0120873939782769, -195.4251063308001903 ) ) ;
#7491=CARTESIAN_POINT ( 'NONE',  ( -73.14859241946263069, -298.6688428153473751, -202.4839277906755797 ) ) ;
#7492=CARTESIAN_POINT ( 'NONE',  ( -9.462182177909394198, -287.0777806097381699, -202.7707827629659221 ) ) ;
#7494=CARTESIAN_POINT ( 'NONE',  ( 10.68516722602901048, -279.7558737880664239, -210.4077516066589624 ) ) ;
#7495=CARTESIAN_POINT ( 'NONE',  ( 35.39271337446832177, -294.5203958933500985, -295.4846725797062277 ) ) ;
#7496=CARTESIAN_POINT ( 'NONE',  ( -7.429742796862990772, -286.8037157253946816, -339.9853298483084814 ) ) ;
#7497=CARTESIAN_POINT ( 'NONE',  ( -37.68462341544178429, -295.3895794750191612, -347.3522851773561229 ) ) ;
#7498=CARTESIAN_POINT ( 'NONE',  ( -57.66489531546407932, -292.1158247085380708, -200.1722482218223433 ) ) ;
#7501=CARTESIAN_POINT ( 'NONE',  ( 65.57626950315574277, 46.04035155596911011, -315.5245225721080828 ) ) ;
#7502=CARTESIAN_POINT ( 'NONE',  ( 37.43278685889510626, -289.2642766528747984, -285.5757113255085642 ) ) ;
#7503=CARTESIAN_POINT ( 'NONE',  ( -72.08107566293803359, -286.9809262143061233, -342.4248175857292154 ) ) ;
#7505=CARTESIAN_POINT ( 'NONE',  ( -59.26513456127775470, -279.1241844158719232, -196.6544303010856254 ) ) ;
#7506=CARTESIAN_POINT ( 'NONE',  ( -54.07545657469196954, -285.2675302851075685, -343.3529032704057045 ) ) ;
#7507=CARTESIAN_POINT ( 'NONE',  ( -113.7367640406030347, -283.1677138658753279, -267.1211478547521097 ) ) ;
#7508=CARTESIAN_POINT ( 'NONE',  ( 2.053330970347486240, -286.6001331627439299, -333.5223855580690611 ) ) ;
#7509=CARTESIAN_POINT ( 'NONE',  ( 34.89226831338478263, -277.7045605732045033, -293.2206736133009031 ) ) ;
#7510=CARTESIAN_POINT ( 'NONE',  ( -75.24792998976515435, -298.0247872125918889, -207.8436233722052577 ) ) ;
#7512=CARTESIAN_POINT ( 'NONE',  ( 24.83559786442586059, -292.7757425721266031, -309.6386536368795532 ) ) ;
#7513=CARTESIAN_POINT ( 'NONE',  ( 15.08576560626180729, -281.4199230255133557, -214.0329021909632274 ) ) ;
#7514=CARTESIAN_POINT ( 'NONE',  ( -94.79085638998031982, -279.1873969923022401, -225.3010778704303902 ) ) ;
#7515=CARTESIAN_POINT ( 'NONE',  ( -68.55930357958888521, -278.9792883320132546, -204.2600294641966627 ) ) ;
#7516=CARTESIAN_POINT ( 'NONE',  ( -27.05166235598578339, -275.2595806962778511, -194.3104845988935381 ) ) ;
#7517=CARTESIAN_POINT ( 'NONE',  ( -80.06543920429247407, -276.5356547595656025, -334.1131574249279765 ) ) ;
#7518=CARTESIAN_POINT ( 'NONE',  ( -49.33571708643257381, -154.2190595633487646, -362.6006225449885960 ) ) ;
#7519=CARTESIAN_POINT ( 'NONE',  ( -101.1263169161629207, -297.4188209467308752, -312.5296757055573948 ) ) ;
#7523=CARTESIAN_POINT ( 'NONE',  ( -96.83369361257679486, -286.2285485655050934, -227.5036289521088122 ) ) ;
#7524=CARTESIAN_POINT ( 'NONE',  ( -65.52266070490216521, -287.4488603876047819, -199.7793967597515916 ) ) ;
#7525=CARTESIAN_POINT ( 'NONE',  ( -42.67962717982778287, -288.4697143638476291, -343.3185769933509164 ) ) ;
#7526=CARTESIAN_POINT ( 'NONE',  ( -55.69358219213990679, -282.7899312403828276, -345.0788222283591153 ) ) ;
#7527=CARTESIAN_POINT ( 'NONE',  ( -106.2540708422838804, -277.3026111395839166, -243.8073779705785853 ) ) ;
#7528=CARTESIAN_POINT ( 'NONE',  ( -110.7155917216020669, -286.2620343397297233, -281.9657661453371702 ) ) ;
#7529=CARTESIAN_POINT ( 'NONE',  ( -68.80187949688786375, -278.1107202179663318, -203.7205532436693716 ) ) ;
#7530=CARTESIAN_POINT ( 'NONE',  ( -101.0016860170209867, -279.3659320730376407, -307.1872531578542862 ) ) ;
#7531=CARTESIAN_POINT ( 'NONE',  ( 22.51985857732192287, -276.6291946196266167, -312.3357182232217042 ) ) ;
#7532=CARTESIAN_POINT ( 'NONE',  ( -69.20620378931118921, -288.2569926970262486, -340.0365204887157802 ) ) ;
#7533=CARTESIAN_POINT ( 'NONE',  ( -76.66644741529918861, -284.3668530391385616, -336.4358553633669544 ) ) ;
#7534=CARTESIAN_POINT ( 'NONE',  ( -35.89406115168510780, -283.5268304124132897, -347.2990659101908477 ) ) ;
#7538=CARTESIAN_POINT ( 'NONE',  ( -18.01616243145861418, -290.6660064438785298, -343.6197630057914125 ) ) ;
#7539=CARTESIAN_POINT ( 'NONE',  ( -99.61981450826766604, -289.8293835929119382, -225.9231303750227369 ) ) ;
#7540=CARTESIAN_POINT ( 'NONE',  ( -62.09799676616633235, -272.7809153287201411, -201.4369986573041444 ) ) ;
#7542=CARTESIAN_POINT ( 'NONE',  ( 26.41304628102256302, -292.3324110308308263, -227.2715612061519437 ) ) ;
#7543=CARTESIAN_POINT ( 'NONE',  ( -26.39079803461989471, -287.3902801190625382, -343.2877873085156466 ) ) ;
#7544=CARTESIAN_POINT ( 'NONE',  ( -1.935229270645188349, -290.7676620133106553, -205.3516790365035263 ) ) ;
#7545=CARTESIAN_POINT ( 'NONE',  ( 35.15382308976920456, -288.9087564804833619, -281.9099528905251759 ) ) ;
#7546=CARTESIAN_POINT ( 'NONE',  ( -106.6662871844225293, -299.4805209788416391, -237.0123917617630980 ) ) ;
#7547=CARTESIAN_POINT ( 'NONE',  ( 24.22491171025234635, -290.1344191207115841, -313.2820103225519119 ) ) ;
#7548=CARTESIAN_POINT ( 'NONE',  ( -96.01611929541947177, -289.1967194168807964, -223.3787705850851353 ) ) ;
#7549=CARTESIAN_POINT ( 'NONE',  ( -111.7136014883612916, -292.6816188629391036, -260.2905747033634611 ) ) ;
#7550=CARTESIAN_POINT ( 'NONE',  ( -92.72924764313725632, -284.8127112288997296, -318.2929105695568524 ) ) ;
#7551=CARTESIAN_POINT ( 'NONE',  ( -53.03209716464139234, -293.8517713624847261, -196.7970998129312648 ) ) ;
#7552=CARTESIAN_POINT ( 'NONE',  ( -113.8396535124608846, -271.2111691839079413, -270.3440440569521002 ) ) ;
#7554=CARTESIAN_POINT ( 'NONE',  ( -99.85839943869147817, -275.0994566530900443, -228.1959883563837082 ) ) ;
#7555=CARTESIAN_POINT ( 'NONE',  ( -24.04615841946317900, -282.0751310521201844, -342.3043615649121421 ) ) ;
#7556=CARTESIAN_POINT ( 'NONE',  ( -29.25361161516740438, -280.9496414997782381, -344.9756191661328444 ) ) ;
#7557=CARTESIAN_POINT ( 'NONE',  ( -112.1148551396041739, -295.9711105592699596, -252.6655221761070038 ) ) ;
#7558=CARTESIAN_POINT ( 'NONE',  ( 19.79522903882365270, -273.1344383052042417, -223.3149136557231316 ) ) ;
#7559=CARTESIAN_POINT ( 'NONE',  ( -111.8330156254960031, -276.6286538162293596, -270.6191118479970896 ) ) ;
#7560=CARTESIAN_POINT ( 'NONE',  ( -93.12961096979383058, -298.5439760193398229, -222.4987571077944608 ) ) ;
#7561=CARTESIAN_POINT ( 'NONE',  ( 34.21650822272301440, -294.7520833863972598, -253.1376664859379275 ) ) ;
#7563=CARTESIAN_POINT ( 'NONE',  ( -67.35211760191585029, -296.2589141621091358, -337.0979870479409328 ) ) ;
#7566=CARTESIAN_POINT ( 'NONE',  ( 32.50801539778480276, -285.9406706493257957, -298.7740774193781590 ) ) ;
#7567=CARTESIAN_POINT ( 'NONE',  ( -93.94254614738427733, -295.8993819926137689, -316.4822198388223455 ) ) ;
#7568=CARTESIAN_POINT ( 'NONE',  ( -111.1079767696223257, -284.2745469950962161, -292.4871306347912423 ) ) ;
#7569=CARTESIAN_POINT ( 'NONE',  ( 37.35733814426770749, -286.9861625435822248, -251.7654740621152882 ) ) ;
#7570=CARTESIAN_POINT ( 'NONE',  ( -30.61749422227395812, -290.1372171988945752, -195.8304968842527956 ) ) ;
#7571=CARTESIAN_POINT ( 'NONE',  ( -3.719015550639384493, -279.6817046848572659, -201.2548502630838811 ) ) ;
#7574=CARTESIAN_POINT ( 'NONE',  ( 35.51653086186653496, -286.4635454192661541, -279.2385433773913519 ) ) ;
#7575=CARTESIAN_POINT ( 'NONE',  ( -67.94321647820565602, -288.3649064124025472, -340.6820942808840300 ) ) ;
#7578=CARTESIAN_POINT ( 'NONE',  ( -96.23051212741820848, -297.5339354342016236, -314.8628036802110159 ) ) ;
#7579=CARTESIAN_POINT ( 'NONE',  ( 18.71545513458323029, -282.2646124421497120, -218.4361563856606381 ) ) ;
#7580=CARTESIAN_POINT ( 'NONE',  ( -100.9149473132007984, -295.1141581088621706, -229.9031268782814550 ) ) ;
#7581=CARTESIAN_POINT ( 'NONE',  ( 17.61797404352745033, -281.9046644720332324, -318.4394052001749174 ) ) ;
#7582=CARTESIAN_POINT ( 'NONE',  ( 21.36902674083426135, -294.3903855568235031, -320.1813001886582697 ) ) ;
#7583=CARTESIAN_POINT ( 'NONE',  ( -96.14510400025876891, -281.1918237686740554, -223.8083484985326663 ) ) ;
#7584=CARTESIAN_POINT ( 'NONE',  ( -70.56360710539951242, -296.6616997712624197, -205.0806829565654539 ) ) ;
#7587=CARTESIAN_POINT ( 'NONE',  ( -43.03373505995562454, -285.1041155077929261, -344.8397983263134847 ) ) ;
#7589=CARTESIAN_POINT ( 'NONE',  ( -4.771743288812454686, -289.9809262143061801, -202.8022627189028810 ) ) ;
#7590=CARTESIAN_POINT ( 'NONE',  ( -60.81205016550025988, -272.9524639128127887, -197.1393481123545826 ) ) ;
#7591=CARTESIAN_POINT ( 'NONE',  ( -104.7022500853002782, -290.7644453777260196, -242.0949726629434622 ) ) ;
#7592=CARTESIAN_POINT ( 'NONE',  ( 23.16499986282335755, -283.6530653494654075, -312.4282905670766013 ) ) ;
#7593=CARTESIAN_POINT ( 'NONE',  ( -93.53604036198451865, -274.8255083754425527, -222.5019076399073583 ) ) ;
#7594=CARTESIAN_POINT ( 'NONE',  ( 30.37562633873334406, -283.6073703194417135, -305.3011252756749627 ) ) ;
#7595=CARTESIAN_POINT ( 'NONE',  ( 35.53212311648148614, -280.4672768188665373, -279.5229458044086641 ) ) ;
#7596=CARTESIAN_POINT ( 'NONE',  ( -36.18438647925570706, -298.0662671119145557, -193.3611179743799084 ) ) ;
#7597=CARTESIAN_POINT ( 'NONE',  ( -7.688617024244204678, -274.2633972671821425, -199.2433162556457376 ) ) ;
#7598=CARTESIAN_POINT ( 'NONE',  ( 27.05030845490103886, -295.9747773250498426, -307.7105949064519450 ) ) ;
#7602=CARTESIAN_POINT ( 'NONE',  ( 31.10381796597688009, -292.1162905066678945, -302.9720514571015997 ) ) ;
#7603=CARTESIAN_POINT ( 'NONE',  ( -14.03988465984631162, -273.8704231777816744, -201.1150795582342425 ) ) ;
#7604=CARTESIAN_POINT ( 'NONE',  ( -71.87595467953094897, -293.1241919154217612, -202.3018618893248401 ) ) ;
#7605=CARTESIAN_POINT ( 'NONE',  ( 39.58706461736021254, -278.0519495502701943, -270.3284710469133074 ) ) ;
#7606=CARTESIAN_POINT ( 'NONE',  ( -53.32154567384359467, -293.0568145391248436, -195.3892560803734852 ) ) ;
#7607=CARTESIAN_POINT ( 'NONE',  ( -51.06324492613408950, -291.2279474053913191, -343.9786727187244537 ) ) ;
#7608=CARTESIAN_POINT ( 'NONE',  ( -68.83150431908634914, -275.4669150004635299, -338.2605629045983164 ) ) ;
#7609=CARTESIAN_POINT ( 'NONE',  ( -59.60278503193910637, -279.2628775725405035, -341.3946191971621147 ) ) ;
#7610=CARTESIAN_POINT ( 'NONE',  ( -9.983073168576796164, -292.7719474781958411, -339.5913117521433264 ) ) ;
#7611=CARTESIAN_POINT ( 'NONE',  ( 23.28124332873744251, -284.0272181631349326, -315.8051958119506821 ) ) ;
#7614=CARTESIAN_POINT ( 'NONE',  ( -1.245244861868627373, -282.2257596511749398, -333.8365731129762821 ) ) ;
#7615=CARTESIAN_POINT ( 'NONE',  ( -31.11263331340023441, -281.2086377712009835, -193.8711398463640876 ) ) ;
#7617=CARTESIAN_POINT ( 'NONE',  ( -88.07013429756909773, -282.5380739131590531, -327.8308650439746543 ) ) ;
#7618=CARTESIAN_POINT ( 'NONE',  ( -114.1492823443344236, -279.4776537539678429, -271.6165480716911134 ) ) ;
#7620=CARTESIAN_POINT ( 'NONE',  ( 33.06626714848160731, -276.6931869621677720, -240.8066092224560748 ) ) ;
#7622=CARTESIAN_POINT ( 'NONE',  ( -109.1418805571601069, -293.0519495502701943, -270.3937649182068412 ) ) ;
#7624=CARTESIAN_POINT ( 'NONE',  ( -47.57004184560806692, -299.9224262388724469, -196.0092313632375465 ) ) ;
#7626=CARTESIAN_POINT ( 'NONE',  ( -105.7895014853543501, -276.1791902067704996, -300.2690069769762431 ) ) ;
#7627=CARTESIAN_POINT ( 'NONE',  ( -110.2660640340680942, -292.5837008754213002, -249.0067000929882965 ) ) ;
#7628=CARTESIAN_POINT ( 'NONE',  ( -0.7140533417946419714, -293.9007257746479240, -333.6826868982256542 ) ) ;
#7629=CARTESIAN_POINT ( 'NONE',  ( -69.33743605679320865, -288.9696059422478811, -340.3455227269321313 ) ) ;
#7631=CARTESIAN_POINT ( 'NONE',  ( 39.06747973268240059, -292.0905341600092697, -267.4770886751508669 ) ) ;
#7632=CARTESIAN_POINT ( 'NONE',  ( 2.900117375362208705, -285.0021159433473485, -208.4980713541659441 ) ) ;
#7633=CARTESIAN_POINT ( 'NONE',  ( -110.4980700321603138, -292.5799634769675208, -257.4571301719701069 ) ) ;
#7634=CARTESIAN_POINT ( 'NONE',  ( -25.00689306722070882, -284.6920396171124139, -197.6556299666691245 ) ) ;
#7635=CARTESIAN_POINT ( 'NONE',  ( -69.20794076186041366, -284.7955577433317558, -336.6002808003874520 ) ) ;
#7636=CARTESIAN_POINT ( 'NONE',  ( -57.21838058625493062, -290.2436529163837236, -344.5627835646071162 ) ) ;
#7637=CARTESIAN_POINT ( 'NONE',  ( 18.00704895523404758, -281.3656396487743905, -222.6501507017215147 ) ) ;
#7638=CARTESIAN_POINT ( 'NONE',  ( 36.70274736358680912, -292.0994463974083715, -250.6781375959988338 ) ) ;
#7639=CARTESIAN_POINT ( 'NONE',  ( -1.866167020558459066, -289.3971126146655024, -338.5200893048668149 ) ) ;
#7640=CARTESIAN_POINT ( 'NONE',  ( 5.528237079389339392, -288.9807012610447714, -334.2492654508545229 ) ) ;
#7641=CARTESIAN_POINT ( 'NONE',  ( -94.95836545548854701, -285.3506306034757358, -225.5153819152156132 ) ) ;
#7644=CARTESIAN_POINT ( 'NONE',  ( -6.282051222323046247, -296.5088506631732344, -339.4668608203849658 ) ) ;
#7645=CARTESIAN_POINT ( 'NONE',  ( -102.7030309332422036, -294.7144204661468621, -310.1253570340539909 ) ) ;
#7646=CARTESIAN_POINT ( 'NONE',  ( -109.1154549935966287, -277.8031526839623666, -255.7401531204066032 ) ) ;
#7647=CARTESIAN_POINT ( 'NONE',  ( -31.25867328258182098, -273.6346691520885770, -193.6502351993405284 ) ) ;
#7648=CARTESIAN_POINT ( 'NONE',  ( -63.83617255819731895, -293.8837330351287846, -339.1811037829581323 ) ) ;
#7649=CARTESIAN_POINT ( 'NONE',  ( 36.36516036808060903, -277.3998447183226403, -277.0896191435438141 ) ) ;
#7650=CARTESIAN_POINT ( 'NONE',  ( 96.73425794709139325, -297.9926885423967065, -196.3887082001726014 ) ) ;
#7651=CARTESIAN_POINT ( 'NONE',  ( 35.68879948544971370, -294.6546769442354616, -262.5444581666731096 ) ) ;
#7652=CARTESIAN_POINT ( 'NONE',  ( -41.04112375576690397, -296.1794408085536361, -343.5894495695878277 ) ) ;
#7654=CARTESIAN_POINT ( 'NONE',  ( -83.09006787485284917, -293.6761491385539102, -330.0683166829167021 ) ) ;
#7655=CARTESIAN_POINT ( 'NONE',  ( -113.3860173099026980, -273.4976330378809735, -258.9787793034378751 ) ) ;
#7656=CARTESIAN_POINT ( 'NONE',  ( -110.4910485170179584, -274.7649140722647303, -253.8029331787696776 ) ) ;
#7657=CARTESIAN_POINT ( 'NONE',  ( -86.87974619603271265, -290.7027659352472710, -324.3686684384343266 ) ) ;
#7658=CARTESIAN_POINT ( 'NONE',  ( -90.41968730244110475, -296.1626224865080985, -320.5818608107164778 ) ) ;
#7659=CARTESIAN_POINT ( 'NONE',  ( -111.1768338370665248, -280.3387799664700424, -285.4839951828166136 ) ) ;
#7660=CARTESIAN_POINT ( 'NONE',  ( -113.5510591164620280, -277.3290768031770881, -263.0443214946834019 ) ) ;
#7663=CARTESIAN_POINT ( 'NONE',  ( -55.68591280941213739, -282.6308908247459613, -345.0391110419173515 ) ) ;
#7664=CARTESIAN_POINT ( 'NONE',  ( 37.49074956737972286, -275.1230969662741472, -288.1214037199364952 ) ) ;
#7665=CARTESIAN_POINT ( 'NONE',  ( -95.42364132032581381, -281.9866027466409264, -316.9410683459303186 ) ) ;
#7666=CARTESIAN_POINT ( 'NONE',  ( -109.7827233945500041, -277.2544304177322942, -246.5561374350880897 ) ) ;
#7667=CARTESIAN_POINT ( 'NONE',  ( -47.83698939556524010, -277.9189514125929463, -195.8782054105980137 ) ) ;
#7669=CARTESIAN_POINT ( 'NONE',  ( -35.78579231260732740, -296.7568535785565587, -196.8683204030683953 ) ) ;
#7670=CARTESIAN_POINT ( 'NONE',  ( 21.35259629559766026, -276.9103621467494918, -223.6506560989280104 ) ) ;
#7672=CARTESIAN_POINT ( 'NONE',  ( 20.95322147525778789, -290.9170975352554365, -222.6106318888103317 ) ) ;
#7673=CARTESIAN_POINT ( 'NONE',  ( -114.1878387977255755, -290.6129992367972363, -265.4958357126591864 ) ) ;
#7674=CARTESIAN_POINT ( 'NONE',  ( 6.152895172813707347, -276.6406331744695990, -208.9927003505397067 ) ) ;
#7675=CARTESIAN_POINT ( 'NONE',  ( -73.71628697692410981, -295.5678831119499819, -204.9629692364338496 ) ) ;
#7676=CARTESIAN_POINT ( 'NONE',  ( -112.3696400062573417, -283.5415057738342739, -286.9432486954008823 ) ) ;
#7678=CARTESIAN_POINT ( 'NONE',  ( -94.00535565743152233, -281.8701695921554915, -319.5152833590767045 ) ) ;
#7680=CARTESIAN_POINT ( 'NONE',  ( -19.96334679007314961, -291.0753015629081233, -198.9985110039530696 ) ) ;
#7681=CARTESIAN_POINT ( 'NONE',  ( -111.4599240142477043, -282.7566209790031735, -265.3587569217504551 ) ) ;
#7684=CARTESIAN_POINT ( 'NONE',  ( 22.60738330158192610, -290.9360399063122031, -225.2933018846084678 ) ) ;
#7685=CARTESIAN_POINT ( 'NONE',  ( -112.7988210684069941, -283.1797209547839316, -258.6585086977402170 ) ) ;
#7686=CARTESIAN_POINT ( 'NONE',  ( -97.52642612285806933, -279.5620666486678374, -313.0941704240725016 ) ) ;
#7687=CARTESIAN_POINT ( 'NONE',  ( -52.11183345544348811, -287.0723337618114783, -195.1415095971085805 ) ) ;
#7688=CARTESIAN_POINT ( 'NONE',  ( -95.76594100401823084, -285.1665145707737565, -226.5934577975501156 ) ) ;
#7689=CARTESIAN_POINT ( 'NONE',  ( -70.70383998876822318, -278.9264471233134941, -335.9533625136695036 ) ) ;
#7690=CARTESIAN_POINT ( 'NONE',  ( -107.9734917034731154, -279.1036162903054674, -289.4333948835920864 ) ) ;
#7691=CARTESIAN_POINT ( 'NONE',  ( -110.5667568546550967, -286.3440450655735958, -286.5812203473781778 ) ) ;
#7693=CARTESIAN_POINT ( 'NONE',  ( -114.1206415309323319, -296.4666736376944982, -263.8683446475938013 ) ) ;
#7695=CARTESIAN_POINT ( 'NONE',  ( 35.30760767710200554, -289.7532316566247914, -287.5053555669150001 ) ) ;
#7697=CARTESIAN_POINT ( 'NONE',  ( 36.57525178469696669, -277.6233781216988064, -234.7283546768995564 ) ) ;
#7699=CARTESIAN_POINT ( 'NONE',  ( 27.38371178845299880, -291.4193583067088866, -230.0486717460100294 ) ) ;
#7700=CARTESIAN_POINT ( 'NONE',  ( -10.51544827116342162, -287.9287060366370383, -201.7103035990886895 ) ) ;
#7701=CARTESIAN_POINT ( 'NONE',  ( -92.98487232703223526, -280.9994775696483771, -221.5380259732319530 ) ) ;
#7702=CARTESIAN_POINT ( 'NONE',  ( 25.85971434397253077, -288.4065610552826229, -227.3937481752561212 ) ) ;
#7703=CARTESIAN_POINT ( 'NONE',  ( 39.11240135817894270, -288.9179131124528226, -274.3802218320415705 ) ) ;
#7704=CARTESIAN_POINT ( 'NONE',  ( -105.9323875721547381, -286.1549196030840108, -300.6978653650383535 ) ) ;
#7705=CARTESIAN_POINT ( 'NONE',  ( -114.3778511503410584, -278.7391516640313398, -268.7363643332592460 ) ) ;
#7707=CARTESIAN_POINT ( 'NONE',  ( 1.016942057057161009, -292.6242209746561684, -335.4604940753806659 ) ) ;
#7708=CARTESIAN_POINT ( 'NONE',  ( 39.27788474882164138, -281.4875186570441770, -278.5206377531734461 ) ) ;
#7709=CARTESIAN_POINT ( 'NONE',  ( -43.60964428983029961, -275.8326859452370741, -196.3394306331634596 ) ) ;
#7711=CARTESIAN_POINT ( 'NONE',  ( 10.59707575819634329, -289.1948066931273615, -210.1954327657594490 ) ) ;
#7712=CARTESIAN_POINT ( 'NONE',  ( -93.38257246444671011, -271.4995230722699375, -219.0253014632682778 ) ) ;
#7714=CARTESIAN_POINT ( 'NONE',  ( -99.51680620269306132, -278.5896029714816109, -231.8947761276758683 ) ) ;
#7715=CARTESIAN_POINT ( 'NONE',  ( 29.59307016885221486, -276.2705804382162569, -232.9996283841600473 ) ) ;
#7716=CARTESIAN_POINT ( 'NONE',  ( 52.55529011099631731, -300.6244180898165723, -196.7495985462560100 ) ) ;
#7717=CARTESIAN_POINT ( 'NONE',  ( -96.99714541536069135, -282.9607609712040812, -318.6937652232096525 ) ) ;
#7718=CARTESIAN_POINT ( 'NONE',  ( -105.6467904554949655, -292.6909565159702993, -241.7252189521745152 ) ) ;
#7719=CARTESIAN_POINT ( 'NONE',  ( -20.71757579726060428, -299.7768269639770438, -194.0502373830632337 ) ) ;
#7721=CARTESIAN_POINT ( 'NONE',  ( -70.57075117558406419, -298.8287550621636797, -201.3405494019295645 ) ) ;
#7723=CARTESIAN_POINT ( 'NONE',  ( -8.501361644253609740, -296.6739735586709799, -339.4276804638399767 ) ) ;
#7724=CARTESIAN_POINT ( 'NONE',  ( -79.42821710171530469, -281.6218152181293704, -332.2380402828636647 ) ) ;
#7725=CARTESIAN_POINT ( 'NONE',  ( -114.0917573914470324, -290.1364766763873604, -276.9475576843412341 ) ) ;
#7726=CARTESIAN_POINT ( 'NONE',  ( -77.42672740886654026, -271.5315811386577707, -207.3925751272192599 ) ) ;
#7727=CARTESIAN_POINT ( 'NONE',  ( -66.89776550876669603, -287.2713448766969577, -200.1266576683457004 ) ) ;
#7728=CARTESIAN_POINT ( 'NONE',  ( -95.20299327749819440, -288.8407391502150290, -315.3958114271890736 ) ) ;
#7729=CARTESIAN_POINT ( 'NONE',  ( -112.5292696805186949, -274.5677371315042024, -270.3867812072841730 ) ) ;
#7730=ORIENTED_EDGE ( 'NONE', *, *, #76024, .T. ) ;
#7731=CARTESIAN_POINT ( 'NONE',  ( -87.01526988795936290, -288.3024077196182020, -328.4921727197404380 ) ) ;
#7732=CARTESIAN_POINT ( 'NONE',  ( 5.853716174388502225, -288.1152533452939792, -329.2989425407670296 ) ) ;
#7734=CARTESIAN_POINT ( 'NONE',  ( -103.7795747657820016, -286.1330110146640777, -231.9475000415241368 ) ) ;
#7735=CARTESIAN_POINT ( 'NONE',  ( 3.149356406875054581, -276.8247395209326100, -331.1275711240854775 ) ) ;
#7736=CARTESIAN_POINT ( 'NONE',  ( 36.41069530732725212, -292.2073198182430360, -249.2876169929024570 ) ) ;
#7737=CARTESIAN_POINT ( 'NONE',  ( -50.06845808036404577, -283.8617499965509978, -346.2525266442955285 ) ) ;
#7738=CARTESIAN_POINT ( 'NONE',  ( 34.66691277832745754, -282.7491219691924584, -244.9553018154132928 ) ) ;
#7739=CARTESIAN_POINT ( 'NONE',  ( -44.41304438088690176, -283.4724330888014379, -347.0678387719418083 ) ) ;
#7740=CARTESIAN_POINT ( 'NONE',  ( 35.05317645576933927, -281.7546275580630777, -260.4423215796209661 ) ) ;
#7741=CARTESIAN_POINT ( 'NONE',  ( 103.4350560888410513, 116.3533902402046039, -283.0411789926872643 ) ) ;
#7742=CARTESIAN_POINT ( 'NONE',  ( 120.4372898702119130, 149.8266080471096870, -262.8568676293995168 ) ) ;
#7743=CARTESIAN_POINT ( 'NONE',  ( -31.73477069997540667, -124.2925422290134208, -360.7507360266465071 ) ) ;
#7744=CARTESIAN_POINT ( 'NONE',  ( -27.25782929498327434, -273.3806123188020933, -197.8468930990040064 ) ) ;
#7745=CARTESIAN_POINT ( 'NONE',  ( -74.58207618928659599, -295.0412269025912337, -337.7459758234620608 ) ) ;
#7746=CARTESIAN_POINT ( 'NONE',  ( -109.3415214902221209, -269.1509101800525627, -295.3710750286876987 ) ) ;
#7747=CARTESIAN_POINT ( 'NONE',  ( -10.50480749357722132, -273.0797659103408819, -198.6592401252945024 ) ) ;
#7748=CARTESIAN_POINT ( 'NONE',  ( -75.87166970081077011, -299.3926353640264892, -206.8483228001516920 ) ) ;
#7749=CARTESIAN_POINT ( 'NONE',  ( -5.564139607152227107, -289.9403148723486652, -336.6289844569672596 ) ) ;
#7751=CARTESIAN_POINT ( 'NONE',  ( -39.09042823831595115, -296.0148425062287174, -347.1059038886952521 ) ) ;
#7752=CARTESIAN_POINT ( 'NONE',  ( -89.71133815167226544, -285.7812382303979462, -219.3433495042972936 ) ) ;
#7753=CARTESIAN_POINT ( 'NONE',  ( -94.84555590992553675, -272.1623599824624762, -219.6186399147071029 ) ) ;
#7754=CARTESIAN_POINT ( 'NONE',  ( 35.33702570241221252, -294.6717908555838221, -295.4633908134493936 ) ) ;
#7755=CARTESIAN_POINT ( 'NONE',  ( 30.84147947820869007, -293.5829467071689010, -234.6012339510699292 ) ) ;
#7756=CARTESIAN_POINT ( 'NONE',  ( -60.26098000395240462, -291.9133906232751769, -200.9993000362906628 ) ) ;
#7758=CARTESIAN_POINT ( 'NONE',  ( -92.14490766997379012, -275.1968761404424981, -218.3237460237761809 ) ) ;
#7759=CARTESIAN_POINT ( 'NONE',  ( 13.71133409898293287, -273.5435252886511535, -213.1798321717830618 ) ) ;
#7761=CARTESIAN_POINT ( 'NONE',  ( -100.4186499674009383, -277.4769843675793481, -314.4159168386735814 ) ) ;
#7763=CARTESIAN_POINT ( 'NONE',  ( 35.81620661834794817, -273.8252641290115434, -260.6471540384591776 ) ) ;
#7764=CARTESIAN_POINT ( 'NONE',  ( -63.42952076588308330, -274.7837419285031615, -201.8373356671743295 ) ) ;
#7765=CARTESIAN_POINT ( 'NONE',  ( 34.34922166516801667, -276.2958808459353577, -255.3393228957438907 ) ) ;
#7766=CARTESIAN_POINT ( 'NONE',  ( -85.18777873020214031, -275.1618072837981117, -211.3295436033829446 ) ) ;
#7768=CARTESIAN_POINT ( 'NONE',  ( 37.91336121491469413, -273.5110305658723746, -265.5700288548729873 ) ) ;
#7769=CARTESIAN_POINT ( 'NONE',  ( -47.79942961734017359, -295.8399312599377708, -342.7625107140514729 ) ) ;
#7770=CARTESIAN_POINT ( 'NONE',  ( -2.883789903580015856, -293.1620033748531000, -335.3844010531342406 ) ) ;
#7772=CARTESIAN_POINT ( 'NONE',  ( -95.86308428181750685, -279.7189087915049868, -220.3931628794002791 ) ) ;
#7773=CARTESIAN_POINT ( 'NONE',  ( 17.28414232958849084, -275.0261739179064762, -221.8608397717020466 ) ) ;
#7774=CARTESIAN_POINT ( 'NONE',  ( -91.54174124195003515, -283.9845055329766410, -216.3643234902861821 ) ) ;
#7775=CARTESIAN_POINT ( 'NONE',  ( -108.1330159686006027, -298.8790747090135369, -245.0902251058344348 ) ) ;
#7777=CARTESIAN_POINT ( 'NONE',  ( -30.50603757819384754, -285.3378227149538588, -197.4687663638026152 ) ) ;
#7778=CARTESIAN_POINT ( 'NONE',  ( -110.4970133349439436, -276.6457991668419822, -281.5982957252188612 ) ) ;
#7779=CARTESIAN_POINT ( 'NONE',  ( -18.88656183603281136, -275.3845748300075797, -341.5986276675744762 ) ) ;
#7780=CARTESIAN_POINT ( 'NONE',  ( -97.41917347918865744, -285.9388096817781388, -315.2787732009737738 ) ) ;
#7781=CARTESIAN_POINT ( 'NONE',  ( 30.53621410309122552, -276.3834113618925130, -242.3042780304308224 ) ) ;
#7783=CARTESIAN_POINT ( 'NONE',  ( 22.14672521501110225, -273.3072902055077407, -222.7214346415330795 ) ) ;
#7784=CARTESIAN_POINT ( 'NONE',  ( -91.76439620766440441, -281.2790824145556030, -218.4388812317861834 ) ) ;
#7786=CARTESIAN_POINT ( 'NONE',  ( -29.10930434397941013, -290.8688905168899623, -345.5238421913936122 ) ) ;
#7787=CARTESIAN_POINT ( 'NONE',  ( 11.41685575594190105, -292.3764198906819729, -327.4164581689026932 ) ) ;
#7790=CARTESIAN_POINT ( 'NONE',  ( -70.63401616881532163, -296.3979187062666369, -204.9349602359829987 ) ) ;
#7791=CARTESIAN_POINT ( 'NONE',  ( -57.97593008291472216, -289.9224807047769445, -198.9975062916075217 ) ) ;
#7792=CARTESIAN_POINT ( 'NONE',  ( 207.9739649226136180, 291.4638663531892462, -68.48153742335392735 ) ) ;
#7794=CARTESIAN_POINT ( 'NONE',  ( -12.46819195455078422, -287.2144499604723933, -342.5553490690209628 ) ) ;
#7795=CARTESIAN_POINT ( 'NONE',  ( -89.17837263452987884, -283.5751211425088059, -214.7293962043702606 ) ) ;
#7796=CARTESIAN_POINT ( 'NONE',  ( -92.99292412680347297, -285.2966533060040319, -318.5291841698085591 ) ) ;
#7797=CARTESIAN_POINT ( 'NONE',  ( -109.7735294940198116, -285.4906532609048213, -260.0542357320898645 ) ) ;
#7798=CARTESIAN_POINT ( 'NONE',  ( -72.38608958492390855, -291.4933863839065111, -337.0861078632919430 ) ) ;
#7799=CARTESIAN_POINT ( 'NONE',  ( -49.72002346270375028, -274.2318256799778737, -194.3302159693817543 ) ) ;
#7800=CARTESIAN_POINT ( 'NONE',  ( -97.19236366976461738, -289.2594414276187536, -224.2184801119245208 ) ) ;
#7801=CARTESIAN_POINT ( 'NONE',  ( 8.241063248432322297, -276.4480114231924404, -332.4852636165502417 ) ) ;
#7802=CARTESIAN_POINT ( 'NONE',  ( 20.99466275004447979, -296.1755330987402886, -316.9509738207449345 ) ) ;
#7804=CARTESIAN_POINT ( 'NONE',  ( -69.91165696735023971, -294.1233781216987495, -202.8022627189028810 ) ) ;
#7805=CARTESIAN_POINT ( 'NONE',  ( -36.20257361892731041, -281.7223979839528738, -343.8454419590273687 ) ) ;
#7806=CARTESIAN_POINT ( 'NONE',  ( -92.01835198473742139, -275.8299030656888817, -322.0157949895496472 ) ) ;
#7807=CARTESIAN_POINT ( 'NONE',  ( -113.4877042674186640, -271.1039975042810397, -264.6586001561869921 ) ) ;
#7808=CARTESIAN_POINT ( 'NONE',  ( 34.80639335941709334, -275.0598188850057682, -282.4372946443554611 ) ) ;
#7809=CARTESIAN_POINT ( 'NONE',  ( 33.97433270854487830, -294.8294560904062109, -251.7941792345553722 ) ) ;
#7810=CARTESIAN_POINT ( 'NONE',  ( 28.61165144478358968, -294.9242566572890496, -302.3146262542020963 ) ) ;
#7811=CARTESIAN_POINT ( 'NONE',  ( 25.99424740338993445, -294.4087614943904896, -227.5227332453404188 ) ) ;
#7812=CARTESIAN_POINT ( 'NONE',  ( 35.90248460558718335, -295.1485931673587402, -292.6447351935624397 ) ) ;
#7813=CARTESIAN_POINT ( 'NONE',  ( -72.12644790865400068, -295.3591005119073998, -334.5549892667825702 ) ) ;
#7814=CARTESIAN_POINT ( 'NONE',  ( -112.1144590672487880, -292.4692947643744105, -276.8270073976423760 ) ) ;
#7815=CARTESIAN_POINT ( 'NONE',  ( -108.2263092204673143, -284.3345099156609876, -300.5702927562213631 ) ) ;
#7816=CARTESIAN_POINT ( 'NONE',  ( 13.15909497732119249, -272.8882905716575920, -213.8111232551791545 ) ) ;
#7817=CARTESIAN_POINT ( 'NONE',  ( 39.57775978659211802, -287.3286859626279579, -265.8205126028088898 ) ) ;
#7818=CARTESIAN_POINT ( 'NONE',  ( -35.04226508535295181, -279.0030212258500910, -344.9704967766186314 ) ) ;
#7819=CARTESIAN_POINT ( 'NONE',  ( -46.76070133416745023, -284.7249658739941083, -197.5198690464767139 ) ) ;
#7820=CARTESIAN_POINT ( 'NONE',  ( 10.81346653292563786, -284.7174067719048480, -212.7948037001758053 ) ) ;
#7821=CARTESIAN_POINT ( 'NONE',  ( -97.57965056221893008, -277.3145912500148142, -224.3868114770451712 ) ) ;
#7822=CARTESIAN_POINT ( 'NONE',  ( -90.78337343436103879, -230.3218577325732781, -348.1307343985224634 ) ) ;
#7823=CARTESIAN_POINT ( 'NONE',  ( -77.07727883789266343, -285.0118166057017675, -208.9898211045761229 ) ) ;
#7825=CARTESIAN_POINT ( 'NONE',  ( 16.93090000069533829, -282.0091973299744268, -216.2266622698892604 ) ) ;
#7826=CARTESIAN_POINT ( 'NONE',  ( -82.72322185915061254, -288.7145941210014257, -332.2750719646207358 ) ) ;
#7827=CARTESIAN_POINT ( 'NONE',  ( -72.45373703409956079, -279.1090686605271003, -338.0039549217130457 ) ) ;
#7828=ADVANCED_FACE ( 'NONE', ( #66291 ), #79375, .T. ) ;
#7829=CARTESIAN_POINT ( 'NONE',  ( -17.46974813775018021, -278.1161131322775759, -344.2421290448695572 ) ) ;
#7830=CARTESIAN_POINT ( 'NONE',  ( -5.556575836668641521, -280.3156372975103636, -204.6442565365026098 ) ) ;
#7832=CARTESIAN_POINT ( 'NONE',  ( 0.2610015416381004649, -276.5353930609064150, -205.8645475316958482 ) ) ;
#7833=CARTESIAN_POINT ( 'NONE',  ( 37.46000585225958446, -293.7812842492056120, -288.6838769745202171 ) ) ;
#7834=CARTESIAN_POINT ( 'NONE',  ( -56.51179552487676006, -287.3203993690483458, -342.5560744034848994 ) ) ;
#7836=CARTESIAN_POINT ( 'NONE',  ( -101.0266835503384186, -292.7091322717921571, -228.4254666199307451 ) ) ;
#7837=CARTESIAN_POINT ( 'NONE',  ( 18.19765951440566099, -293.1512774009930240, -318.2300770456562304 ) ) ;
#7838=CARTESIAN_POINT ( 'NONE',  ( 34.50474111316298576, -293.0459148747185623, -257.2464007213786772 ) ) ;
#7839=CARTESIAN_POINT ( 'NONE',  ( -106.9855132839358305, -292.0456940053614971, -238.1217449781401001 ) ) ;
#7840=CARTESIAN_POINT ( 'NONE',  ( 32.83011356680909643, -281.9328945366125936, -249.8718712637184467 ) ) ;
#7841=CARTESIAN_POINT ( 'NONE',  ( -36.17635543328511716, -296.9867554724299907, -193.6704353362449922 ) ) ;
#7842=CARTESIAN_POINT ( 'NONE',  ( -17.74229264157356312, -289.4571983152096095, -344.7195473127935088 ) ) ;
#7843=CARTESIAN_POINT ( 'NONE',  ( -19.23689546071541301, -280.9613325135925379, -343.9850312482377035 ) ) ;
#7844=CARTESIAN_POINT ( 'NONE',  ( 12.40539572523971401, -288.7142162585620326, -329.1060815590088851 ) ) ;
#7845=CARTESIAN_POINT ( 'NONE',  ( -77.06412516446302163, -285.8373119732323744, -209.0294615953273194 ) ) ;
#7847=CARTESIAN_POINT ( 'NONE',  ( -49.42433641670088207, -154.1833738735614077, -363.2467176495409831 ) ) ;
#7848=CARTESIAN_POINT ( 'NONE',  ( 201.9871895515904043, 292.2036489450776457, -53.99999999998372147 ) ) ;
#7849=CARTESIAN_POINT ( 'NONE',  ( -79.13876353550847398, -278.6691146984443321, -210.3144093544044608 ) ) ;
#7850=CARTESIAN_POINT ( 'NONE',  ( -71.07170645813098986, -278.5164105010307480, -205.2584726204851222 ) ) ;
#7851=CARTESIAN_POINT ( 'NONE',  ( -31.25750281044283696, -273.7937095030862906, -193.6097999099276592 ) ) ;
#7852=CARTESIAN_POINT ( 'NONE',  ( -106.8576566752619783, -266.2287397320313289, -305.9886098359324933 ) ) ;
#7853=CARTESIAN_POINT ( 'NONE',  ( -72.22152776909865679, -278.1746721828476439, -202.3612588296030026 ) ) ;
#7854=CARTESIAN_POINT ( 'NONE',  ( -54.08253899494208383, -281.2881180102810958, -343.1577038242150479 ) ) ;
#7855=CARTESIAN_POINT ( 'NONE',  ( 28.70513694042041308, -295.8079305119152878, -308.0412502057671986 ) ) ;
#7856=CARTESIAN_POINT ( 'NONE',  ( -9.710012036928262091, -292.9153293096463244, -202.6724007151781564 ) ) ;
#7857=CARTESIAN_POINT ( 'NONE',  ( -29.13456773689200219, -287.6307889366717632, -343.3945791871334450 ) ) ;
#7858=CARTESIAN_POINT ( 'NONE',  ( -15.81385885964917470, -274.9748115644696327, -196.4826544351321616 ) ) ;
#7859=CARTESIAN_POINT ( 'NONE',  ( -93.08102006560196173, -296.0486911266057177, -317.5199371560336203 ) ) ;
#7863=CARTESIAN_POINT ( 'NONE',  ( -109.9602055073348765, -280.7390416093109025, -249.4836929548602029 ) ) ;
#7864=CARTESIAN_POINT ( 'NONE',  ( -34.31426914201708911, -281.1707443673003013, -197.1019463498369078 ) ) ;
#7865=CARTESIAN_POINT ( 'NONE',  ( -109.6948069130452694, -280.0145456464238691, -293.7467858612341161 ) ) ;
#7866=CARTESIAN_POINT ( 'NONE',  ( 29.52441060181652333, -281.0133473354478042, -300.3575081863629634 ) ) ;
#7867=CARTESIAN_POINT ( 'NONE',  ( -4.986337434218993003, -272.9659516091461455, -204.1366003303986929 ) ) ;
#7870=CARTESIAN_POINT ( 'NONE',  ( 38.56648807445828453, -276.2045202652068383, -258.3555646900310308 ) ) ;
#7872=CARTESIAN_POINT ( 'NONE',  ( 15.56298187118347265, -278.3045312282047234, -323.5946947879721165 ) ) ;
#7873=CARTESIAN_POINT ( 'NONE',  ( -92.91799830677950922, -276.4046985153819946, -322.8763751534348216 ) ) ;
#7875=DIRECTION ( 'NONE',  ( 0.000000000000000000, 0.000000000000000000, -1.000000000000000000 ) ) ;
#7876=CARTESIAN_POINT ( 'NONE',  ( -110.9136329199378537, -286.3237800610236263, -286.6576670865500205 ) ) ;
#7877=CARTESIAN_POINT ( 'NONE',  ( -92.67193276102551636, -290.4298858457653409, -222.4949808486858274 ) ) ;
#7878=CARTESIAN_POINT ( 'NONE',  ( 22.01678789598922847, -286.2430670753387858, -221.4746915785638635 ) ) ;
#7879=CARTESIAN_POINT ( 'NONE',  ( -94.21492683277554647, -282.1291721564969066, -317.7257683049259640 ) ) ;
#7880=CARTESIAN_POINT ( 'NONE',  ( -98.02848019283301539, -282.5510825744433419, -312.0731454985016171 ) ) ;
#7881=CARTESIAN_POINT ( 'NONE',  ( 19.78221980405417568, -284.9674739533084562, -222.6110511891691317 ) ) ;
#7882=CARTESIAN_POINT ( 'NONE',  ( 34.33146479532327078, -282.9647166658353967, -286.1752868207253186 ) ) ;
#7883=CARTESIAN_POINT ( 'NONE',  ( -69.25692826692680626, -271.6322069577688580, -202.4764768922208020 ) ) ;
#7885=CARTESIAN_POINT ( 'NONE',  ( -109.4740261224480093, -282.6392924544429093, -294.9246674279370382 ) ) ;
#7886=CARTESIAN_POINT ( 'NONE',  ( -112.3648795842791941, -298.5256188982440335, -272.4404370897309491 ) ) ;
#7888=CARTESIAN_POINT ( 'NONE',  ( -68.63467242439438110, -280.5716956690453685, -204.1481409026625897 ) ) ;
#7889=CARTESIAN_POINT ( 'NONE',  ( -70.28624685163519814, -287.6191410373857593, -202.7986633752721275 ) ) ;
#7893=CARTESIAN_POINT ( 'NONE',  ( 35.31267797015716781, -295.2066607720008733, -249.5617856799250660 ) ) ;
#7895=CARTESIAN_POINT ( 'NONE',  ( -107.1381010420987394, -276.1947112032342488, -297.8103996846610926 ) ) ;
#7896=CARTESIAN_POINT ( 'NONE',  ( -23.35139513059944960, -288.0749500300123032, -345.9692720543474707 ) ) ;
#7897=CARTESIAN_POINT ( 'NONE',  ( 22.46485579483354300, -291.3534596134875301, -227.1005611582333472 ) ) ;
#7898=CARTESIAN_POINT ( 'NONE',  ( -108.9706615412812596, -277.0207249879943561, -286.8649032456038412 ) ) ;
#7899=CARTESIAN_POINT ( 'NONE',  ( -87.33907527759036782, -293.8978430308621910, -325.2348635833365051 ) ) ;
#7900=CARTESIAN_POINT ( 'NONE',  ( -92.94047739810316955, -292.5475500958058319, -222.2984563303981247 ) ) ;
#7901=CARTESIAN_POINT ( 'NONE',  ( 35.77081079830085031, -277.8376638359845288, -253.6410175316879361 ) ) ;
#7902=CARTESIAN_POINT ( 'NONE',  ( -27.85341573640096513, -293.4137773554000432, -346.1283948010387803 ) ) ;
#7903=CARTESIAN_POINT ( 'NONE',  ( 35.75556045586952791, -289.2860665322921818, -280.6135695641382881 ) ) ;
#7904=CARTESIAN_POINT ( 'NONE',  ( -113.1040745153595992, -288.7098464367003317, -276.8445238061522673 ) ) ;
#7905=CARTESIAN_POINT ( 'NONE',  ( 3.960202679077717836, -289.9094446596550370, -331.3284650955091024 ) ) ;
#7907=CARTESIAN_POINT ( 'NONE',  ( -78.25627047467871478, -290.4206444389456578, -331.0735626091944823 ) ) ;
#7909=CARTESIAN_POINT ( 'NONE',  ( -15.05304048304508058, -289.9749397069415977, -343.7052226039473339 ) ) ;
#7910=CARTESIAN_POINT ( 'NONE',  ( -87.81075411548221155, -277.3710099016477670, -214.4032642897158780 ) ) ;
#7911=CARTESIAN_POINT ( 'NONE',  ( -106.1585801564188785, -279.3306217380792873, -235.7462808467416835 ) ) ;
#7912=CARTESIAN_POINT ( 'NONE',  ( 30.70510843258561451, -280.7527074191285124, -234.2561307284209988 ) ) ;
#7913=CARTESIAN_POINT ( 'NONE',  ( 36.98155252631730860, -285.4180333054229095, -259.9282364223599302 ) ) ;
#7915=CARTESIAN_POINT ( 'NONE',  ( -24.64217692196449860, -278.3554982582028288, -197.2202430342596529 ) ) ;
#7916=CARTESIAN_POINT ( 'NONE',  ( -78.09490476767805944, -281.5999099516347428, -333.3228282422173265 ) ) ;
#7918=CARTESIAN_POINT ( 'NONE',  ( -98.26169566711723746, -276.4143253438988381, -316.3332161561735347 ) ) ;
#7919=CARTESIAN_POINT ( 'NONE',  ( -104.1545026975579020, -282.9807547602968611, -308.1189680917823921 ) ) ;
#7920=CARTESIAN_POINT ( 'NONE',  ( -65.88555339742242722, -274.4717160403345133, -202.9975509168688745 ) ) ;
#7921=CARTESIAN_POINT ( 'NONE',  ( -92.28220072421791542, -292.8499697486639661, -221.0676545624600635 ) ) ;
#7922=CARTESIAN_POINT ( 'NONE',  ( -23.48784656349971200, -299.5373519014282806, -193.8512418494217684 ) ) ;
#7923=CARTESIAN_POINT ( 'NONE',  ( 26.65710265469163076, -274.7374777641269930, -235.0955074956486897 ) ) ;
#7924=CARTESIAN_POINT ( 'NONE',  ( -9.730641833557097442, -296.6916292594438573, -340.0936793098232442 ) ) ;
#7925=CARTESIAN_POINT ( 'NONE',  ( -28.97506936117078169, -289.1156991169128787, -346.9587456471790574 ) ) ;
#7926=CARTESIAN_POINT ( 'NONE',  ( 18.12012216225994266, -278.9197260147113866, -219.0454238271456120 ) ) ;
#7927=CARTESIAN_POINT ( 'NONE',  ( -33.53724234021917994, -291.9321216610143210, -193.4551617408098991 ) ) ;
#7929=CARTESIAN_POINT ( 'NONE',  ( -94.29480758823179087, -288.9618003250732841, -316.4018825239820671 ) ) ;
#7930=CARTESIAN_POINT ( 'NONE',  ( 22.41950978074509493, -292.1718727155264901, -315.6777643980386188 ) ) ;
#7933=CARTESIAN_POINT ( 'NONE',  ( -110.3986519023002302, -290.0490111061756124, -271.1797991876197784 ) ) ;
#7935=CARTESIAN_POINT ( 'NONE',  ( -57.70509259614949826, -286.7368315208547642, -196.2913908803028846 ) ) ;
#7936=CARTESIAN_POINT ( 'NONE',  ( -105.5937364680635966, -293.2662352645559167, -254.8156830097664738 ) ) ;
#7937=CARTESIAN_POINT ( 'NONE',  ( -36.28973329757899080, -294.0980555643682237, -347.1316803670979994 ) ) ;
#7938=EDGE_CURVE ( 'NONE', #8402, #38700, #69074, .T. ) ;
#7939=CARTESIAN_POINT ( 'NONE',  ( 39.03799595980812853, -282.9333955015293895, -275.6102689358332896 ) ) ;
#7940=CARTESIAN_POINT ( 'NONE',  ( -85.72456080356995756, -285.1937654039052177, -215.6300524162169552 ) ) ;
#7941=CARTESIAN_POINT ( 'NONE',  ( 17.64344766955986898, -276.1744823984302002, -221.5222512166006936 ) ) ;
#7942=CARTESIAN_POINT ( 'NONE',  ( -25.98140794945219412, -292.9268743664404155, -344.1363886498006082 ) ) ;
#7943=CARTESIAN_POINT ( 'NONE',  ( 35.41613615781426461, -274.2202530623489452, -260.6953141466017314 ) ) ;
#7946=CARTESIAN_POINT ( 'NONE',  ( 15.46109875539708689, -293.9964709504282041, -326.3754797260445457 ) ) ;
#7947=CARTESIAN_POINT ( 'NONE',  ( -14.13994448591539310, -288.2754540701741348, -199.5752238779358265 ) ) ;
#7948=CARTESIAN_POINT ( 'NONE',  ( -76.91091064297273761, -296.6483323364652733, -336.1174144921039328 ) ) ;
#7950=CARTESIAN_POINT ( 'NONE',  ( 33.12531798419511375, -287.9469192570459768, -250.9113872191048813 ) ) ;
#7951=CARTESIAN_POINT ( 'NONE',  ( -112.8364222513997248, -277.4355549987857330, -284.3390504998582173 ) ) ;
#7952=CARTESIAN_POINT ( 'NONE',  ( -19.30313127504841475, -295.4775053082207705, -345.1683424128270303 ) ) ;
#7953=CARTESIAN_POINT ( 'NONE',  ( -23.56025265417988379, -287.0175368800004776, -344.9152156619758784 ) ) ;
#7954=CARTESIAN_POINT ( 'NONE',  ( 35.46780223414203448, -294.2023151367526452, -295.5149038562099122 ) ) ;
#7956=CARTESIAN_POINT ( 'NONE',  ( -6.036413579860385070, -292.8085834472713032, -204.3771384064993697 ) ) ;
#7959=CARTESIAN_POINT ( 'NONE',  ( -21.04059066060629135, -109.3119883924524771, -359.1154128302550816 ) ) ;
#7960=CARTESIAN_POINT ( 'NONE',  ( -2.556400534608909147, -288.0238275467715994, -202.4297073922786865 ) ) ;
#7961=CARTESIAN_POINT ( 'NONE',  ( -19.05039376806006857, -283.7666405000204009, -190.3683826091709363 ) ) ;
#7962=EDGE_LOOP ( 'NONE', ( #25311, #79005, #28023, #91449 ) ) ;
#7964=CARTESIAN_POINT ( 'NONE',  ( -112.3005092421667115, -278.1156456214510513, -253.2004151000520267 ) ) ;
#7965=CARTESIAN_POINT ( 'NONE',  ( -96.55178080688489217, -285.9235182833341469, -316.1443998227013594 ) ) ;
#7966=CARTESIAN_POINT ( 'NONE',  ( -103.9126535757035015, -282.6352095054799065, -307.9771861908458845 ) ) ;
#7968=CARTESIAN_POINT ( 'NONE',  ( -10.22183121759466573, -286.7753876966069697, -339.7404668137065187 ) ) ;
#7969=CARTESIAN_POINT ( 'NONE',  ( -35.57669818200841405, -275.9344558797519653, -194.6039557898241696 ) ) ;
#7970=CARTESIAN_POINT ( 'NONE',  ( -107.8967211018427008, -297.2954636387335654, -251.3398210208746093 ) ) ;
#7971=CARTESIAN_POINT ( 'NONE',  ( 23.33070614837535928, -292.8112814322578856, -311.9242032630952508 ) ) ;
#7972=CARTESIAN_POINT ( 'NONE',  ( 20.98336255574975695, -281.5260210089689394, -220.2262317231332247 ) ) ;
#7973=CARTESIAN_POINT ( 'NONE',  ( 33.58653086281132971, -275.7806169780106984, -287.6818394754311043 ) ) ;
#7974=CARTESIAN_POINT ( 'NONE',  ( -83.49568151612434974, -278.7486767383157371, -213.6060776626616189 ) ) ;
#7975=CARTESIAN_POINT ( 'NONE',  ( -41.19106775703900780, -275.0845710428190500, -193.7148463023310114 ) ) ;
#7976=CARTESIAN_POINT ( 'NONE',  ( -6.710842559334417423, -275.5797089320426494, -340.6835161545515120 ) ) ;
#7977=CARTESIAN_POINT ( 'NONE',  ( -48.55409767859317327, -154.7049544282948546, -365.0407483515516560 ) ) ;
#7978=CARTESIAN_POINT ( 'NONE',  ( -26.80725467259023986, -274.9181422207075798, -344.6694346137963976 ) ) ;
#7979=CARTESIAN_POINT ( 'NONE',  ( -112.8104714642036157, -298.1292117583039385, -258.3168843575630262 ) ) ;
#7980=CARTESIAN_POINT ( 'NONE',  ( -69.85430415644619018, -279.9805209788416391, -337.9475929042657754 ) ) ;
#7981=CARTESIAN_POINT ( 'NONE',  ( 202.9739649223127742, 291.4636489454787807, -68.19743562414970484 ) ) ;
#7982=CARTESIAN_POINT ( 'NONE',  ( -89.89400091338661980, -286.3684677463857611, -219.1758144907784640 ) ) ;
#7983=CARTESIAN_POINT ( 'NONE',  ( -32.39507036174258303, -287.8738255240219814, -194.5226353243144217 ) ) ;
#7984=CARTESIAN_POINT ( 'NONE',  ( 19.59981007584344681, -286.2532955138565853, -224.4985394635234002 ) ) ;
#7985=CARTESIAN_POINT ( 'NONE',  ( -106.0196446601928102, -276.5946788698287264, -297.3755650157638115 ) ) ;
#7986=CARTESIAN_POINT ( 'NONE',  ( -95.23363775000161979, -285.7665605741071317, -316.8505576613182484 ) ) ;
#7987=CARTESIAN_POINT ( 'NONE',  ( -96.15348774456148817, -277.6502049444628710, -225.9343076109350932 ) ) ;
#7988=CARTESIAN_POINT ( 'NONE',  ( -97.27824057330747110, -279.2771582993402717, -312.9135989107572868 ) ) ;
#7990=CARTESIAN_POINT ( 'NONE',  ( 34.22610807783807019, -276.2382313293148286, -285.0593243508667456 ) ) ;
#7991=CARTESIAN_POINT ( 'NONE',  ( 38.95060028379592154, -286.4337139448103926, -277.2526791771106787 ) ) ;
#7992=CARTESIAN_POINT ( 'NONE',  ( -5.021231372576554719, -281.2697649534921993, -200.6506731364722498 ) ) ;
#7993=CARTESIAN_POINT ( 'NONE',  ( 37.80677678180712320, -282.2517723688818592, -286.9214769481020539 ) ) ;
#7996=DIRECTION ( 'NONE',  ( -0.8510748438184358999, -0.5250018354872690862, -0.006684530980050039546 ) ) ;
#7997=CARTESIAN_POINT ( 'NONE',  ( 15.83615169445521254, -290.1695175808054614, -324.4009525675751320 ) ) ;
#7998=CARTESIAN_POINT ( 'NONE',  ( -112.1541873705144781, -289.4392702276746832, -254.2871902977917387 ) ) ;
#7999=CARTESIAN_POINT ( 'NONE',  ( -8.669945598421884725, -296.2834264217712530, -341.0170974821744494 ) ) ;
#8000=CARTESIAN_POINT ( 'NONE',  ( -44.57489798370398404, -297.1555933027912602, -197.5075850789002345 ) ) ;
#8001=CARTESIAN_POINT ( 'NONE',  ( -2.095157989460947778, -291.8549465728301584, -202.0016882125615609 ) ) ;
#8002=CARTESIAN_POINT ( 'NONE',  ( 20.90040732358131947, -285.4021005891712548, -225.2106509410555759 ) ) ;
#8004=CARTESIAN_POINT ( 'NONE',  ( -0.7803967397976755427, -289.7604347740268622, -334.0623913322140766 ) ) ;
#8005=CARTESIAN_POINT ( 'NONE',  ( -106.6662871844225293, -293.4805209788415823, -237.0123917617630980 ) ) ;
#8006=CARTESIAN_POINT ( 'NONE',  ( 35.21617955764460817, -289.7962630860748732, -289.3441300505067488 ) ) ;
#8007=CARTESIAN_POINT ( 'NONE',  ( 2.193668350929908417, -286.5242751726996175, -334.3516811274839142 ) ) ;
#8008=CARTESIAN_POINT ( 'NONE',  ( -40.78026240149577575, -291.0955449567578626, -345.2948692940261708 ) ) ;
#8009=CARTESIAN_POINT ( 'NONE',  ( -101.9732587860497546, -285.0242763615592025, -304.9098380994175841 ) ) ;
#8010=CARTESIAN_POINT ( 'NONE',  ( -83.16926140034645698, -293.4268758796561656, -210.7147740084812710 ) ) ;
#8012=CARTESIAN_POINT ( 'NONE',  ( -73.18521390427548567, -275.5596664071740634, -204.0184947702227589 ) ) ;
#8013=CARTESIAN_POINT ( 'NONE',  ( -34.85126290705520091, -282.2172706411769241, -343.4926593903437606 ) ) ;
#8014=CARTESIAN_POINT ( 'NONE',  ( -6.452414031569595032, -280.6463450089007665, -338.7188412135294016 ) ) ;
#8015=CARTESIAN_POINT ( 'NONE',  ( -0.7920108885427427081, -293.7765922506057450, -337.9650164259404050 ) ) ;
#8016=CARTESIAN_POINT ( 'NONE',  ( -79.41291222442505671, -271.7156659612984981, -209.4056313917288605 ) ) ;
#8017=CARTESIAN_POINT ( 'NONE',  ( 12.69795933561254131, -274.4281117527275455, -325.5431708728868898 ) ) ;
#8018=CARTESIAN_POINT ( 'NONE',  ( -108.9613680081086358, -298.0833784048866733, -253.8727386661447838 ) ) ;
#8020=CARTESIAN_POINT ( 'NONE',  ( -111.2830537992627740, -295.0139568837859656, -252.8496864380457794 ) ) ;
#8022=CARTESIAN_POINT ( 'NONE',  ( -35.61876750191357388, -296.4554241701134174, -343.9427735942774120 ) ) ;
#8024=CARTESIAN_POINT ( 'NONE',  ( -72.19251452969369609, -296.3284564878208585, -334.7028803549815166 ) ) ;
#8026=CARTESIAN_POINT ( 'NONE',  ( -98.00479789158495691, -283.1801664615961727, -225.5718821187446679 ) ) ;
#8027=CARTESIAN_POINT ( 'NONE',  ( -105.9871871336933395, -296.2195411300162391, -295.3451539059549305 ) ) ;
#8028=CARTESIAN_POINT ( 'NONE',  ( -95.81656071533025454, -285.2288055099918438, -220.1843345743191662 ) ) ;
#8029=CARTESIAN_POINT ( 'NONE',  ( -2.280207228873084802, -284.5119467509238689, -337.2939643009593738 ) ) ;
#8030=CARTESIAN_POINT ( 'NONE',  ( 20.27374764682814146, -286.5264429128648658, -219.2314271746945451 ) ) ;
#8031=CARTESIAN_POINT ( 'NONE',  ( -41.67413367338352970, -289.9974237825621799, -195.6021983822802213 ) ) ;
#8033=CARTESIAN_POINT ( 'NONE',  ( -8.911334228678228442, -279.6119048896013055, -198.9757335164242988 ) ) ;
#8034=CARTESIAN_POINT ( 'NONE',  ( -54.49178911615187815, -274.7666405000204009, -345.3538533559490702 ) ) ;
#8037=CARTESIAN_POINT ( 'NONE',  ( 34.39551870740162798, -286.5514388889804991, -285.9410210727103276 ) ) ;
#8038=CARTESIAN_POINT ( 'NONE',  ( -77.98429921428237321, -288.5046875320861091, -335.4589974825216814 ) ) ;
#8039=CARTESIAN_POINT ( 'NONE',  ( 82.64890176555634582, -299.5541904835127980, -188.7068768330456123 ) ) ;
#8040=CARTESIAN_POINT ( 'NONE',  ( -96.75637080641293153, -298.7593735611004035, -226.5637852109154551 ) ) ;
#8041=CARTESIAN_POINT ( 'NONE',  ( -105.8092805577969528, -279.5367008895115646, -304.4035007314972177 ) ) ;
#8042=CARTESIAN_POINT ( 'NONE',  ( -58.41602785233541084, -293.3432175373289965, -342.7638291730453943 ) ) ;
#8043=CARTESIAN_POINT ( 'NONE',  ( -5.545452586470449141, -280.1490631427390099, -204.6261491367922360 ) ) ;
#8044=CARTESIAN_POINT ( 'NONE',  ( 13.39742235110125534, -294.5320294081415113, -328.3502179017373805 ) ) ;
#8046=CARTESIAN_POINT ( 'NONE',  ( 15.31355574053964475, -284.8689055239517529, -216.1694375706188964 ) ) ;
#8047=CARTESIAN_POINT ( 'NONE',  ( -109.8862592678147507, -280.3071135819704409, -289.4453676147621763 ) ) ;
#8049=CARTESIAN_POINT ( 'NONE',  ( -96.28258130028333994, -296.2184039834166924, -226.8729404565453365 ) ) ;
#8053=CARTESIAN_POINT ( 'NONE',  ( 35.66881769675151759, -283.3308813288306851, -254.7661243090953462 ) ) ;
#8055=CARTESIAN_POINT ( 'NONE',  ( -69.85430415644619018, -295.1237833571632905, -202.7746430608542312 ) ) ;
#8056=CARTESIAN_POINT ( 'NONE',  ( 21.73328103353280127, -274.0870780364297161, -221.2255359479905223 ) ) ;
#8057=CARTESIAN_POINT ( 'NONE',  ( -95.11308969468898056, -291.0137705497180036, -225.7352672671156029 ) ) ;
#8058=CARTESIAN_POINT ( 'NONE',  ( 27.47396739210304872, -283.5462114003387342, -305.4272981945176753 ) ) ;
#8059=CARTESIAN_POINT ( 'NONE',  ( -2.554364777748514115, -276.1205098279206709, -205.2743934086977617 ) ) ;
#8061=CARTESIAN_POINT ( 'NONE',  ( 37.08855623747116681, -283.3593742402736098, -286.7486451572592614 ) ) ;
#8062=CARTESIAN_POINT ( 'NONE',  ( 26.81331540313337314, -279.8622380372074758, -234.7063218668481568 ) ) ;
#8063=CARTESIAN_POINT ( 'NONE',  ( -26.71359343580094503, -278.9171112211891455, -344.6042590453749881 ) ) ;
#8065=CARTESIAN_POINT ( 'NONE',  ( -46.87889485985060389, -273.7675372613273908, -193.9540376748857682 ) ) ;
#8066=CARTESIAN_POINT ( 'NONE',  ( 35.48130958705406357, -295.6727240364586464, -285.8536021694327474 ) ) ;
#8069=CARTESIAN_POINT ( 'NONE',  ( 115.2940338803257703, -299.5541904835127980, -195.3611179825600175 ) ) ;
#8070=CARTESIAN_POINT ( 'NONE',  ( 36.25441539508127420, -291.9211693323629788, -288.4130340596161659 ) ) ;
#8071=CARTESIAN_POINT ( 'NONE',  ( -27.27550220494214628, -273.6910477003168012, -197.9454051131689596 ) ) ;
#8074=CARTESIAN_POINT ( 'NONE',  ( -56.03781801345316183, -293.3358651313317864, -196.3258327148124067 ) ) ;
#8075=CARTESIAN_POINT ( 'NONE',  ( 10.59707575819634329, -283.1948066931273047, -210.1954327657594490 ) ) ;
#8076=CARTESIAN_POINT ( 'NONE',  ( 6.257574296360926880, -293.8349236778196314, -207.3761039925192051 ) ) ;
#8077=CARTESIAN_POINT ( 'NONE',  ( -17.97508163599090736, -290.8022013000285710, -342.6989315005793628 ) ) ;
#8078=CARTESIAN_POINT ( 'NONE',  ( -21.28384270088205099, -274.8456881282380664, -343.5045865777364611 ) ) ;
#8079=CARTESIAN_POINT ( 'NONE',  ( -97.23738653589296632, -279.8644862052773306, -314.5845220144026939 ) ) ;
#8080=CARTESIAN_POINT ( 'NONE',  ( 6.899508285148374220, -292.5250614885724190, -330.2921079519918521 ) ) ;
#8081=CARTESIAN_POINT ( 'NONE',  ( 0.7324147085716452565, -282.4142087380836301, -204.7982106011602070 ) ) ;
#8083=CARTESIAN_POINT ( 'NONE',  ( -58.95843874355288960, -283.0062483690753083, -340.1624237813173295 ) ) ;
#8084=CARTESIAN_POINT ( 'NONE',  ( -92.85951881761224058, -280.3587417919036966, -217.3771528269134592 ) ) ;
#8086=CARTESIAN_POINT ( 'NONE',  ( -27.43871699845037782, -281.7240578219924600, -346.3743220323171954 ) ) ;
#8087=CARTESIAN_POINT ( 'NONE',  ( 3.386854982995440633, -277.4605135324746357, -335.4929283865736807 ) ) ;
#8089=CARTESIAN_POINT ( 'NONE',  ( 29.33222022470513934, -276.5855759547884531, -233.1405731757521380 ) ) ;
#8090=CARTESIAN_POINT ( 'NONE',  ( -102.0172624299486870, -286.6233781216988064, -301.5434626090942061 ) ) ;
#8092=CARTESIAN_POINT ( 'NONE',  ( -55.81014109018446590, -299.8146850886207631, -197.6168102559092006 ) ) ;
#8094=CARTESIAN_POINT ( 'NONE',  ( -32.33486341200443803, -275.0089483619669295, -344.8889075913206170 ) ) ;
#8095=CARTESIAN_POINT ( 'NONE',  ( -53.20001070164216372, -293.6117907162477536, -195.9938901986680833 ) ) ;
#8096=CARTESIAN_POINT ( 'NONE',  ( -30.78958769864947342, -291.4857469110150987, -197.5534089751789395 ) ) ;
#8097=CARTESIAN_POINT ( 'NONE',  ( -20.51597483970617475, -288.3494539409715571, -345.4918477423779564 ) ) ;
#8099=CARTESIAN_POINT ( 'NONE',  ( 37.48859745676208632, -291.9312284321855486, -254.8362292020100028 ) ) ;
#8100=CARTESIAN_POINT ( 'NONE',  ( -76.56943090731783741, -281.9860072957666830, -332.9325681215935901 ) ) ;
#8101=CARTESIAN_POINT ( 'NONE',  ( -99.12578378033575177, -291.8504972091675995, -311.5375296093928910 ) ) ;
#8102=CARTESIAN_POINT ( 'NONE',  ( -109.4020804703804117, -282.8296436716500466, -285.8486754552714046 ) ) ;
#8103=CARTESIAN_POINT ( 'NONE',  ( 22.99917629516962947, -283.4481504871378093, -312.3161190070868543 ) ) ;
#8104=CARTESIAN_POINT ( 'NONE',  ( -37.48906997160655408, -289.9951653540702523, -347.1387154300267639 ) ) ;
#8106=CARTESIAN_POINT ( 'NONE',  ( -34.31705220668383305, -280.5835150816415648, -197.3496601180021628 ) ) ;
#8107=CARTESIAN_POINT ( 'NONE',  ( 24.50300054096744873, -291.7438655633978328, -225.1588866379612455 ) ) ;
#8108=CARTESIAN_POINT ( 'NONE',  ( 18.22763561303820268, -287.6270598464529940, -217.2164403377509814 ) ) ;
#8109=CARTESIAN_POINT ( 'NONE',  ( -14.96415025754044947, -289.2623259260079180, -344.0291359362524872 ) ) ;
#8110=CARTESIAN_POINT ( 'NONE',  ( -7.018441519922675731, -286.6281392526678360, -203.9433253405669859 ) ) ;
#8113=CARTESIAN_POINT ( 'NONE',  ( 38.01124758832005313, -295.5189946042634119, -278.7344361196631439 ) ) ;
#8115=CARTESIAN_POINT ( 'NONE',  ( -37.70356343775669927, -293.7413911527011692, -346.8801077522113019 ) ) ;
#8116=CARTESIAN_POINT ( 'NONE',  ( -109.2766588292207075, -277.4293624597767121, -284.1667998989694297 ) ) ;
#8117=CARTESIAN_POINT ( 'NONE',  ( -34.04404987219109557, -297.4410138449539431, -193.4634035313384004 ) ) ;
#8118=CARTESIAN_POINT ( 'NONE',  ( 31.48276417105896030, -291.6835363480417982, -244.0191198579662455 ) ) ;
#8119=CARTESIAN_POINT ( 'NONE',  ( -0.05486954881660670996, -276.3156775524662407, -206.4114672360272493 ) ) ;
#8120=CARTESIAN_POINT ( 'NONE',  ( -88.81459125358490780, -295.5575627746709984, -217.1057959254890193 ) ) ;
#8121=CARTESIAN_POINT ( 'NONE',  ( 36.01771416011681026, -294.7263899151772648, -268.0101949775855132 ) ) ;
#8122=CARTESIAN_POINT ( 'NONE',  ( 11.12490944502650869, -293.8214164374300026, -215.2914478877239617 ) ) ;
#8125=CARTESIAN_POINT ( 'NONE',  ( -98.53128193849934746, -293.9586314598638523, -314.1050217684543782 ) ) ;
#8126=CARTESIAN_POINT ( 'NONE',  ( -105.3926320780602168, -298.1367108294285231, -302.0119830350562324 ) ) ;
#8127=CARTESIAN_POINT ( 'NONE',  ( -88.81796530879852014, -290.7383936896437717, -322.4533685666158362 ) ) ;
#8128=CARTESIAN_POINT ( 'NONE',  ( -41.03604514216881682, -295.4331711629549204, -343.3013195127070958 ) ) ;
#8129=CARTESIAN_POINT ( 'NONE',  ( -97.47530550890830625, -279.9137734892112235, -315.7954604370450511 ) ) ;
#8130=CARTESIAN_POINT ( 'NONE',  ( -98.17399215065155715, -277.8597449689636392, -223.9422556973289886 ) ) ;
#8132=CARTESIAN_POINT ( 'NONE',  ( 19.96545856242100925, -274.2037152016761183, -219.0071071626609296 ) ) ;
#8133=CARTESIAN_POINT ( 'NONE',  ( -23.82759904544685270, -280.9579894241214220, -343.5641457005611414 ) ) ;
#8134=CARTESIAN_POINT ( 'NONE',  ( -88.38035010239748601, -277.7507125657219831, -213.7793486349378611 ) ) ;
#8135=CARTESIAN_POINT ( 'NONE',  ( 19.69207575226213436, -278.8748759124342200, -221.3805653360641372 ) ) ;
#8137=CARTESIAN_POINT ( 'NONE',  ( -100.3107428087508168, -295.7561046765929405, -232.3657085698484366 ) ) ;
#8138=CARTESIAN_POINT ( 'NONE',  ( -36.30535200196021606, -276.0652672355307686, -195.3556616230930274 ) ) ;
#8140=CARTESIAN_POINT ( 'NONE',  ( -103.1608118071919051, -289.0583347044720881, -233.6698201309343403 ) ) ;
#8141=CARTESIAN_POINT ( 'NONE',  ( -48.86899637170681387, -289.1949671333656511, -346.5473251627266791 ) ) ;
#8142=CARTESIAN_POINT ( 'NONE',  ( -3.408529488362511461, -276.4991874036045374, -203.2753996071324138 ) ) ;
#8143=CARTESIAN_POINT ( 'NONE',  ( -97.88107605473174999, -271.1564458993732387, -226.0031569106832876 ) ) ;
#8144=CARTESIAN_POINT ( 'NONE',  ( -110.0751358337139010, -283.4364597119254086, -295.1402654811672619 ) ) ;
#8146=CARTESIAN_POINT ( 'NONE',  ( 23.93971589769808617, -278.9643665410040967, -227.1004771850872999 ) ) ;
#8148=CARTESIAN_POINT ( 'NONE',  ( -28.04090243351973655, -290.9676184676383741, -197.5046971835992338 ) ) ;
#8149=CARTESIAN_POINT ( 'NONE',  ( -99.12212090931139130, -283.2536217067654434, -229.2023389870147696 ) ) ;
#8152=CARTESIAN_POINT ( 'NONE',  ( 5.670939392648947752, -290.6342601277420954, -208.8571153759386902 ) ) ;
#8153=CARTESIAN_POINT ( 'NONE',  ( -98.29824191064153638, -279.5797322628210395, -311.9632865491652751 ) ) ;
#8154=CARTESIAN_POINT ( 'NONE',  ( -67.70975448991417522, -284.6469725979753207, -340.6874288034358642 ) ) ;
#8155=CARTESIAN_POINT ( 'NONE',  ( -12.36568005723957775, -274.8097769455103503, -341.7287714476520364 ) ) ;
#8156=CARTESIAN_POINT ( 'NONE',  ( -91.52122179960639414, -285.2535121589745586, -221.3626210168351065 ) ) ;
#8157=CARTESIAN_POINT ( 'NONE',  ( 36.28869640350418990, -276.9933397310216492, -271.5767323975772456 ) ) ;
#8158=CARTESIAN_POINT ( 'NONE',  ( -66.85845467276556064, -278.2519756885929496, -337.3041006508607325 ) ) ;
#8159=CARTESIAN_POINT ( 'NONE',  ( -109.9326084848987506, -286.3094202279793308, -289.2682818673715133 ) ) ;
#8163=CARTESIAN_POINT ( 'NONE',  ( -112.1206950522465462, -270.5523142621871102, -270.3356552556181214 ) ) ;
#8164=CARTESIAN_POINT ( 'NONE',  ( -92.69847972270899561, -295.6522570676820578, -323.8833279277232009 ) ) ;
#8165=CARTESIAN_POINT ( 'NONE',  ( 20.81039032277737988, -290.1790772233784992, -317.1604895947701834 ) ) ;
#8167=CARTESIAN_POINT ( 'NONE',  ( -72.02372285203398405, -279.9805209788415823, -342.4524372437778652 ) ) ;
#8168=CARTESIAN_POINT ( 'NONE',  ( -82.04747367213400366, -278.3785845518816586, -208.0483077362997051 ) ) ;
#8169=CARTESIAN_POINT ( 'NONE',  ( 12.76787395916058365, -291.1376611916884372, -212.9549249512255358 ) ) ;
#8171=CARTESIAN_POINT ( 'NONE',  ( -14.36806484283705920, -287.8754864141963594, -200.2867486383720745 ) ) ;
#8172=CARTESIAN_POINT ( 'NONE',  ( -110.9086939320789043, -280.2008211621055125, -278.9290772286676088 ) ) ;
#8173=CARTESIAN_POINT ( 'NONE',  ( 37.97298062650322947, -288.8139260698100657, -257.3883140021017653 ) ) ;
#8174=CARTESIAN_POINT ( 'NONE',  ( -93.13631810824165314, -285.8538830937043258, -320.4999047093288596 ) ) ;
#8175=CARTESIAN_POINT ( 'NONE',  ( -69.01343525507078880, -277.6239253166676235, -340.5602870983317985 ) ) ;
#8176=CARTESIAN_POINT ( 'NONE',  ( -73.62481522715789595, -295.5881481331142595, -205.1278261547325599 ) ) ;
#8177=CARTESIAN_POINT ( 'NONE',  ( 38.21697244273757832, -291.5957320311709395, -267.5156877626960750 ) ) ;
#8178=CARTESIAN_POINT ( 'NONE',  ( -112.0854050171260781, -278.6175655975350196, -251.8035534840315961 ) ) ;
#8180=CARTESIAN_POINT ( 'NONE',  ( -100.3410428545005004, -274.9454999920176306, -231.0934685075681045 ) ) ;
#8183=CARTESIAN_POINT ( 'NONE',  ( -37.37352853689063892, -294.5519495502701943, -195.3611179825600175 ) ) ;
#8184=CARTESIAN_POINT ( 'NONE',  ( -38.32156247796196169, -272.2798927552709642, -194.3807660033862419 ) ) ;
#8186=CARTESIAN_POINT ( 'NONE',  ( -74.53171740694234870, -279.0509903461343697, -207.4150453568209684 ) ) ;
#8188=CARTESIAN_POINT ( 'NONE',  ( 16.68611286523719173, -277.5095746022453795, -324.7399367696779677 ) ) ;
#8189=CARTESIAN_POINT ( 'NONE',  ( -50.07355810752827807, -299.3117679249257890, -197.8816401418131079 ) ) ;
#8190=CARTESIAN_POINT ( 'NONE',  ( -67.79905309717629791, -282.5009917377072952, -340.8250794350179831 ) ) ;
#8191=CARTESIAN_POINT ( 'NONE',  ( 34.69242566093825531, -289.5335162531466722, -287.3628454926237055 ) ) ;
#8192=CARTESIAN_POINT ( 'NONE',  ( -110.1574025285620451, -298.3635507047486612, -247.3695676159385641 ) ) ;
#8193=CARTESIAN_POINT ( 'NONE',  ( -9.306518152596988003, -299.6008830229522459, -193.7525902071232906 ) ) ;
#8194=CARTESIAN_POINT ( 'NONE',  ( 21.99201416585045976, -296.1785539566021725, -315.9840673755689409 ) ) ;
#8195=CARTESIAN_POINT ( 'NONE',  ( -4.033465500463715436, -280.6116839055916330, -337.3729821306352505 ) ) ;
#8196=CARTESIAN_POINT ( 'NONE',  ( -72.66429445132308729, -271.6025235429034410, -204.5451790722492262 ) ) ;
#8197=CARTESIAN_POINT ( 'NONE',  ( 24.87996056931854127, -288.5637787123874318, -226.3510703271207092 ) ) ;
#8200=CARTESIAN_POINT ( 'NONE',  ( -3.234759334076432236, -287.5112433257053226, -335.3091091258291385 ) ) ;
#8201=CARTESIAN_POINT ( 'NONE',  ( 191.2182377077906210, 270.1866636230031986, -139.4034682273137093 ) ) ;
#8203=CARTESIAN_POINT ( 'NONE',  ( -51.59333685379478140, -287.8057490131084251, -345.4310663107943355 ) ) ;
#8204=CARTESIAN_POINT ( 'NONE',  ( 14.09526769726614326, -287.9718319416722352, -322.1908954051531850 ) ) ;
#8206=CARTESIAN_POINT ( 'NONE',  ( -110.6347129470287598, -285.9184972853026920, -247.6073563475782748 ) ) ;
#8207=CARTESIAN_POINT ( 'NONE',  ( -90.98049828805513073, -278.1733347450403357, -319.9822838292565166 ) ) ;
#8209=CARTESIAN_POINT ( 'NONE',  ( -2.185239688717064421, -291.4267576358827228, -202.1883777198423502 ) ) ;
#8210=CARTESIAN_POINT ( 'NONE',  ( 31.92603756300851359, -281.7731774274238887, -236.8426344075677150 ) ) ;
#8211=CARTESIAN_POINT ( 'NONE',  ( 38.83832826753946676, -283.1383104555060868, -275.5938904056896490 ) ) ;
#8212=CARTESIAN_POINT ( 'NONE',  ( -4.169101813171855575, -282.9599755698355921, -339.8401485919889069 ) ) ;
#8213=CARTESIAN_POINT ( 'NONE',  ( -37.01249035395545661, -280.3896690971016596, -197.3407159855634632 ) ) ;
#8214=CARTESIAN_POINT ( 'NONE',  ( 203.7385753312324255, 295.8239488676054521, -68.68380676480988711 ) ) ;
#8215=CARTESIAN_POINT ( 'NONE',  ( -67.51919413461016006, -279.4491100218172051, -338.8399270025230408 ) ) ;
#8216=CARTESIAN_POINT ( 'NONE',  ( 102.1048073347433984, 116.7066834670583688, -282.3738722355800519 ) ) ;
#8217=CARTESIAN_POINT ( 'NONE',  ( -40.39622826133777522, -139.3177327926281919, -361.3465267510854346 ) ) ;
#8218=CARTESIAN_POINT ( 'NONE',  ( -48.89086778907831388, -273.0985731122017341, -198.0656734554658556 ) ) ;
#8219=CARTESIAN_POINT ( 'NONE',  ( 39.65004385586741620, -293.0592443801769491, -270.3162576741946737 ) ) ;
#8220=CARTESIAN_POINT ( 'NONE',  ( 199.4771156391817044, 285.7106110358174647, -96.36288505241603275 ) ) ;
#8221=CARTESIAN_POINT ( 'NONE',  ( -60.70449132435135908, -272.4402049955682514, -197.4534070751128922 ) ) ;
#8222=CARTESIAN_POINT ( 'NONE',  ( -109.4487032702568996, -288.7462267643866198, -286.1368280742186130 ) ) ;
#8223=CARTESIAN_POINT ( 'NONE',  ( -47.94645742184883375, -297.0487392896868641, -343.8870997488448893 ) ) ;
#8224=CARTESIAN_POINT ( 'NONE',  ( 31.86941091889186595, -289.1942513318580836, -295.0808587808870698 ) ) ;
#8226=CARTESIAN_POINT ( 'NONE',  ( -41.91951042189564447, -296.0496237935923318, -347.0414396277783453 ) ) ;
#8227=CARTESIAN_POINT ( 'NONE',  ( -72.40905352599041578, -286.0671283506696341, -206.2511077312405803 ) ) ;
#8228=CARTESIAN_POINT ( 'NONE',  ( -68.70502247561516640, -272.5698384764476145, -200.3622514046079743 ) ) ;
#8229=CARTESIAN_POINT ( 'NONE',  ( 37.91451346131207600, -294.5494031122284468, -285.8743748071310051 ) ) ;
#8230=CARTESIAN_POINT ( 'NONE',  ( 26.43837157476315269, -293.4759869089399444, -227.2368466991587184 ) ) ;
#8231=CARTESIAN_POINT ( 'NONE',  ( -30.80908708362613169, -292.3037082016740555, -197.6540002339139903 ) ) ;
#8233=CARTESIAN_POINT ( 'NONE',  ( -1.997142436358078532, -276.4366632153182763, -203.5773142433344844 ) ) ;
#8234=CARTESIAN_POINT ( 'NONE',  ( 36.20896316335802823, -274.0751114480273145, -248.7674764491355006 ) ) ;
#8236=CARTESIAN_POINT ( 'NONE',  ( -103.3555684037344236, -278.5766898961941820, -230.7392407679122073 ) ) ;
#8237=CARTESIAN_POINT ( 'NONE',  ( -33.98411455798402869, -272.4949557075995585, -196.6375326412457412 ) ) ;
#8238=CARTESIAN_POINT ( 'NONE',  ( -107.4963497813586883, -273.9143837811582785, -248.9138678115826053 ) ) ;
#8239=CARTESIAN_POINT ( 'NONE',  ( -51.61902788433417300, -274.8064208554403649, -198.4790382186501745 ) ) ;
#8240=CARTESIAN_POINT ( 'NONE',  ( -23.56068614086864343, -299.8220829685578792, -194.1574325805405294 ) ) ;
#8241=CARTESIAN_POINT ( 'NONE',  ( 33.19127283596517941, -273.2293864945604582, -243.8374205445818745 ) ) ;
#8242=CARTESIAN_POINT ( 'NONE',  ( -100.2499685906837072, -296.6914469935880447, -307.6957334255300225 ) ) ;
#8243=CARTESIAN_POINT ( 'NONE',  ( 34.34532835409838469, -292.3450716859035197, -287.0401950425402902 ) ) ;
#8245=CARTESIAN_POINT ( 'NONE',  ( 10.49270609881256355, -276.9043465753118198, -330.6902227387937501 ) ) ;
#8246=CARTESIAN_POINT ( 'NONE',  ( -6.530911435774659601, -274.6351094645378907, -204.1818515564873167 ) ) ;
#8247=CARTESIAN_POINT ( 'NONE',  ( -103.6049059239891648, -283.7385512346713767, -232.0133426163484671 ) ) ;
#8248=CARTESIAN_POINT ( 'NONE',  ( -106.1064065531918033, -298.9505159643125580, -239.8770417912992059 ) ) ;
#8250=CARTESIAN_POINT ( 'NONE',  ( -97.48286507373671839, -284.3287431583534044, -228.6779405996006460 ) ) ;
#8252=CARTESIAN_POINT ( 'NONE',  ( -98.82303473716640951, -277.3576158127910958, -229.0631199027758385 ) ) ;
#8253=CARTESIAN_POINT ( 'NONE',  ( -56.77309693657972645, -275.8822281979100808, -341.3914749303068561 ) ) ;
#8254=CARTESIAN_POINT ( 'NONE',  ( -40.64440112943640315, -285.0938264587467756, -345.3010594970865554 ) ) ;
#8255=CARTESIAN_POINT ( 'NONE',  ( 36.09638666303445831, -276.7731785992814935, -271.5763092790903102 ) ) ;
#8257=CARTESIAN_POINT ( 'NONE',  ( 36.80861786471962205, -274.1745353556555074, -287.9720487661896868 ) ) ;
#8258=CARTESIAN_POINT ( 'NONE',  ( -87.72198962451302862, -281.3504217467373678, -214.5771162053004559 ) ) ;
#8260=CARTESIAN_POINT ( 'NONE',  ( -77.77297098924006491, -287.4338113103829073, -206.5283165921237583 ) ) ;
#8262=CARTESIAN_POINT ( 'NONE',  ( 2.156387640704739095, -290.5804653806386568, -206.5443217577132202 ) ) ;
#8265=CARTESIAN_POINT ( 'NONE',  ( -84.31726006802928453, -296.1842205489926982, -213.8994950413990921 ) ) ;
#8266=CARTESIAN_POINT ( 'NONE',  ( -110.9212095917192613, -288.8243750878549463, -260.1358897349019799 ) ) ;
#8267=CARTESIAN_POINT ( 'NONE',  ( 6.757860130087521178, -59.91093500391586701, -350.7441993381422094 ) ) ;
#8268=CARTESIAN_POINT ( 'NONE',  ( -35.73738983254033030, -296.0720782082398728, -195.3616562271829764 ) ) ;
#8269=CARTESIAN_POINT ( 'NONE',  ( -48.78431811421492625, -287.6750899408974078, -345.8584267106271000 ) ) ;
#8270=CARTESIAN_POINT ( 'NONE',  ( -33.43370511856519300, -284.6023051227076621, -344.0702867015227184 ) ) ;
#8271=CARTESIAN_POINT ( 'NONE',  ( -64.16819136358799369, -283.9468019447569986, -199.2534442105668404 ) ) ;
#8272=CARTESIAN_POINT ( 'NONE',  ( 18.06033515703222392, -283.6629337773714497, -318.7965327575103061 ) ) ;
#8273=CARTESIAN_POINT ( 'NONE',  ( -106.3225653737429894, -285.0294912301480394, -294.8889956474224050 ) ) ;
#8274=CARTESIAN_POINT ( 'NONE',  ( -88.35899231476878413, -291.7427507734794290, -325.8195952284083319 ) ) ;
#8275=CARTESIAN_POINT ( 'NONE',  ( -85.79821248650144128, -273.7351768733041126, -210.5471505377111896 ) ) ;
#8276=CARTESIAN_POINT ( 'NONE',  ( 9.319132046145174542, -286.4969820008562351, -329.8589765446868114 ) ) ;
#8277=CARTESIAN_POINT ( 'NONE',  ( 16.02703672096978949, -274.7840385955083775, -214.8563620859998196 ) ) ;
#8278=CARTESIAN_POINT ( 'NONE',  ( 35.82380454034149864, -295.3412768050098407, -255.5741056924946122 ) ) ;
#8280=CARTESIAN_POINT ( 'NONE',  ( -4.771743288812468897, -291.1233781216987495, -337.9199732462171255 ) ) ;
#8281=CARTESIAN_POINT ( 'NONE',  ( -71.65386404591605185, -282.2003801067847917, -335.3528011916450851 ) ) ;
#8282=CARTESIAN_POINT ( 'NONE',  ( -64.45805579246368211, -275.4049527938127540, -340.5212201520491817 ) ) ;
#8283=CARTESIAN_POINT ( 'NONE',  ( -92.65611466045429268, -271.7571550717036075, -217.7775872492336475 ) ) ;
#8284=CARTESIAN_POINT ( 'NONE',  ( 33.33863155232842246, -275.1467891088194619, -289.0207905950664440 ) ) ;
#8285=CARTESIAN_POINT ( 'NONE',  ( -41.65256892093166385, -293.5171378067259411, -196.7436581752837128 ) ) ;
#8286=CARTESIAN_POINT ( 'NONE',  ( 4.628708955301119587, -293.5751990842128976, -210.2831850550282411 ) ) ;
#8287=CARTESIAN_POINT ( 'NONE',  ( -107.9458880956823350, -286.0220183876300553, -292.5652314561752974 ) ) ;
#8288=CARTESIAN_POINT ( 'NONE',  ( 37.18255999887779240, -294.7640880704538517, -253.4282480202897432 ) ) ;
#8289=CARTESIAN_POINT ( 'NONE',  ( 29.03939691517057398, -294.3699160090109217, -232.3236597731639677 ) ) ;
#8290=CARTESIAN_POINT ( 'NONE',  ( -101.4683276015983182, -295.9093519217059907, -305.2434294506728065 ) ) ;
#8291=CARTESIAN_POINT ( 'NONE',  ( -83.76479713648667769, -291.6896254559972590, -329.2669471489276702 ) ) ;
#8292=CARTESIAN_POINT ( 'NONE',  ( -113.1365919914083804, -284.5454640079326509, -284.2234378506873895 ) ) ;
#8293=CARTESIAN_POINT ( 'NONE',  ( 96.03965234238681603, -297.7891995914106928, -194.8443227416307195 ) ) ;
#8294=CARTESIAN_POINT ( 'NONE',  ( -69.79090538727119508, -285.4699400018363349, -200.5180403070917521 ) ) ;
#8295=CARTESIAN_POINT ( 'NONE',  ( -104.6024050281223907, -280.1023295313847825, -302.8510595676843877 ) ) ;
#8296=CARTESIAN_POINT ( 'NONE',  ( -71.34864170662183369, -284.3874575923714474, -205.3176061596872159 ) ) ;
#8297=CARTESIAN_POINT ( 'NONE',  ( 35.20324031050567726, -285.7965889188588449, -289.3935184728280774 ) ) ;
#8298=CARTESIAN_POINT ( 'NONE',  ( -42.32477241687654157, -278.1295268111490486, -194.7603608983119727 ) ) ;
#8300=CARTESIAN_POINT ( 'NONE',  ( -109.0410930147352104, -283.8747183874442044, -284.4033934928929739 ) ) ;
#8301=CARTESIAN_POINT ( 'NONE',  ( 14.87936773103877997, -281.9734963913975321, -214.2442732148389837 ) ) ;
#8302=CARTESIAN_POINT ( 'NONE',  ( -89.34092821436455267, -288.8220770088713039, -326.8314685290400234 ) ) ;
#8303=CARTESIAN_POINT ( 'NONE',  ( -90.75359746618231327, -279.3940657768375218, -324.7821109420657990 ) ) ;
#8304=CARTESIAN_POINT ( 'NONE',  ( 0.8157055774802070003, -277.8698426935357020, -336.7334363566346838 ) ) ;
#8305=CARTESIAN_POINT ( 'NONE',  ( -66.06774586248181436, -279.4987798963685464, -203.2370157507219801 ) ) ;
#8306=CARTESIAN_POINT ( 'NONE',  ( -91.40490094741399218, -275.2580322838123834, -218.8738074127771256 ) ) ;
#8307=CARTESIAN_POINT ( 'NONE',  ( 37.76130585578759735, -293.3390465869196078, -253.3155804573571288 ) ) ;
#8308=CARTESIAN_POINT ( 'NONE',  ( -42.80900180664941246, -287.1414497675957023, -344.8571732011448603 ) ) ;
#8309=CARTESIAN_POINT ( 'NONE',  ( -106.5425496607384304, -292.5660672429578995, -238.3341873027603981 ) ) ;
#8310=CARTESIAN_POINT ( 'NONE',  ( 17.30183688811230525, -293.1688335152245486, -319.2503779049449122 ) ) ;
#8311=CARTESIAN_POINT ( 'NONE',  ( -26.20836917106474928, -294.5732202134387876, -342.5285374217200456 ) ) ;
#8312=CARTESIAN_POINT ( 'NONE',  ( -113.5048797576731801, -291.5135498281408104, -279.7800091927238668 ) ) ;
#8313=CARTESIAN_POINT ( 'NONE',  ( 4.975421513624708858, -281.2926752247358877, -210.7527806139052302 ) ) ;
#8315=CARTESIAN_POINT ( 'NONE',  ( -3.565874001828468920, -297.3860441556971068, -193.6762481238071416 ) ) ;
#8316=CARTESIAN_POINT ( 'NONE',  ( -8.263978578098019057, -289.3326826881709053, -341.5638405283590373 ) ) ;
#8317=CARTESIAN_POINT ( 'NONE',  ( -76.14596299181764039, -281.7040340603282402, -335.4952581766779076 ) ) ;
#8318=CARTESIAN_POINT ( 'NONE',  ( -43.17645838374929212, -289.4572102199495021, -347.1185273162600993 ) ) ;
#8319=CARTESIAN_POINT ( 'NONE',  ( 13.15111011125132556, -287.1145974696386247, -217.5413515927343155 ) ) ;
#8320=CARTESIAN_POINT ( 'NONE',  ( 201.7240241516389574, 293.7293971981536629, -83.18315247025914516 ) ) ;
#8321=CARTESIAN_POINT ( 'NONE',  ( 63.22103669990880803, 47.92133741242891176, -316.8191042900280081 ) ) ;
#8322=CARTESIAN_POINT ( 'NONE',  ( -55.60814623013595792, -169.4418122124796753, -360.5495281866856772 ) ) ;
#8323=CARTESIAN_POINT ( 'NONE',  ( -110.5123360852229837, -277.7818060068988757, -267.8926382502700108 ) ) ;
#8324=CARTESIAN_POINT ( 'NONE',  ( -107.5190650318384940, -277.7519552007705670, -249.1629216190852105 ) ) ;
#8325=CARTESIAN_POINT ( 'NONE',  ( -1.307633499101990004, -274.1835922031394830, -202.3369286543063481 ) ) ;
#8326=CARTESIAN_POINT ( 'NONE',  ( 175.0041629047781271, 240.4131245324038844, -177.6887199834764317 ) ) ;
#8327=CARTESIAN_POINT ( 'NONE',  ( -113.6445838756358029, -277.0757253824085637, -274.4202094164843402 ) ) ;
#8328=CARTESIAN_POINT ( 'NONE',  ( -2.413054757375911574, -296.3565715061034780, -337.8441806628794097 ) ) ;
#8330=CARTESIAN_POINT ( 'NONE',  ( 8.882930851629504687, -293.1981947323657778, -213.7157178095656889 ) ) ;
#8331=CARTESIAN_POINT ( 'NONE',  ( -73.84358200006384720, -274.5211940095080081, -202.7710458423248667 ) ) ;
#8332=CARTESIAN_POINT ( 'NONE',  ( -0.7604210395519718224, -287.2405917456084694, -334.1617750186446756 ) ) ;
#8333=CARTESIAN_POINT ( 'NONE',  ( -105.5224101039212172, -273.6642203059287226, -234.6833361348515723 ) ) ;
#8334=CARTESIAN_POINT ( 'NONE',  ( -84.07646283080694616, -297.5557556038510256, -214.2160486507111727 ) ) ;
#8337=CARTESIAN_POINT ( 'NONE',  ( -110.3461926727412248, -280.7214898202737459, -250.8262824034354708 ) ) ;
#8338=CARTESIAN_POINT ( 'NONE',  ( -59.84152288778496143, -280.8334954296590809, -200.5366440328770068 ) ) ;
#8339=CARTESIAN_POINT ( 'NONE',  ( -113.2005444345684992, -280.3681265287311248, -265.9554679596756159 ) ) ;
#8340=CARTESIAN_POINT ( 'NONE',  ( 19.54630740871675343, -273.3744187275711397, -223.5160290947762576 ) ) ;
#8343=CARTESIAN_POINT ( 'NONE',  ( -22.19647948440641727, -280.4181250650603943, -198.8976211804902903 ) ) ;
#8344=CARTESIAN_POINT ( 'NONE',  ( 24.34411847373105431, -275.7445173515255306, -224.5460701886739514 ) ) ;
#8345=CARTESIAN_POINT ( 'NONE',  ( 13.54539285635240731, -278.3402571773850127, -325.5272365306250322 ) ) ;
#8346=CARTESIAN_POINT ( 'NONE',  ( -111.6068383973752987, -276.8995921752079994, -288.3963945737141898 ) ) ;
#8349=CARTESIAN_POINT ( 'NONE',  ( 21.26040569712759165, -284.1812917122802560, -317.7544739925014596 ) ) ;
#8350=CARTESIAN_POINT ( 'NONE',  ( -70.28429003828244959, -290.8035571044527501, -205.0358740298112252 ) ) ;
#8351=CARTESIAN_POINT ( 'NONE',  ( -18.19937023769119833, -285.6410405840448448, -195.8286810658755428 ) ) ;
#8352=CARTESIAN_POINT ( 'NONE',  ( -95.08954205613500221, -282.1465896852297419, -316.6755718151316614 ) ) ;
#8353=CARTESIAN_POINT ( 'NONE',  ( 5.923989895202256939, -281.0270416693567199, -329.8880445152174730 ) ) ;
#8354=CARTESIAN_POINT ( 'NONE',  ( -8.921422392047762884, -284.5066286355018406, -201.5461639253691715 ) ) ;
#8355=CARTESIAN_POINT ( 'NONE',  ( -67.48330849950752963, -280.8528163151304966, -203.4249888109294773 ) ) ;
#8357=CARTESIAN_POINT ( 'NONE',  ( -4.526998554563204991, -281.0268790313537011, -339.1478018420622789 ) ) ;
#8358=CARTESIAN_POINT ( 'NONE',  ( -25.20566982056843841, -296.8977247283833094, -344.4253852945511198 ) ) ;
#8359=CARTESIAN_POINT ( 'NONE',  ( -97.07067353381347630, -278.9032966661787896, -312.7604598173548993 ) ) ;
#8360=CARTESIAN_POINT ( 'NONE',  ( -65.22161571679001213, -287.6888408989054824, -200.5422930956303276 ) ) ;
#8363=CARTESIAN_POINT ( 'NONE',  ( 128.9467878515196162, -299.5541904835127980, -195.3611179825600175 ) ) ;
#8364=CARTESIAN_POINT ( 'NONE',  ( -2.737519560770817595, -294.4260979987192854, -203.1762019396395544 ) ) ;
#8365=CARTESIAN_POINT ( 'NONE',  ( 6.547080839558873322, -274.4559378005754411, -331.2427951825577566 ) ) ;
#8366=CARTESIAN_POINT ( 'NONE',  ( 28.75961725698642013, -287.2608121016148175, -309.5373181568937184 ) ) ;
#8367=CARTESIAN_POINT ( 'NONE',  ( -9.405963006380487101, -290.8231915656431852, -201.9983542393699736 ) ) ;
#8368=CARTESIAN_POINT ( 'NONE',  ( -93.99683139834648671, -276.5776266211051393, -317.1936558139399267 ) ) ;
#8369=CARTESIAN_POINT ( 'NONE',  ( -100.9430361440342381, -295.2109505874921069, -231.9762781301447774 ) ) ;
#8370=CARTESIAN_POINT ( 'NONE',  ( -109.1962319081563635, -292.0695460811627413, -254.9283689660583150 ) ) ;
#8373=CARTESIAN_POINT ( 'NONE',  ( -93.19529745392752318, -294.3167414348046691, -322.3715539003737831 ) ) ;
#8374=CARTESIAN_POINT ( 'NONE',  ( 13.67805720154488291, -288.3812406307868059, -216.9668605901659362 ) ) ;
#8375=CARTESIAN_POINT ( 'NONE',  ( -106.3308848451127204, -289.2063383509611185, -238.3851461425439879 ) ) ;
#8376=CARTESIAN_POINT ( 'NONE',  ( 33.65517424816048475, -289.2333833429689207, -289.9106266486477921 ) ) ;
#8377=DIRECTION ( 'NONE',  ( -1.000000000000000000, -0.000000000000000000, -0.000000000000000000 ) ) ;
#8378=CARTESIAN_POINT ( 'NONE',  ( -26.44075465362175237, -289.7128606397769204, -342.7570880605549064 ) ) ;
#8380=CARTESIAN_POINT ( 'NONE',  ( 0.5363793263533368494, -289.7644264455269649, -337.0037948326392439 ) ) ;
#8381=CARTESIAN_POINT ( 'NONE',  ( -74.18133490481001502, -277.5851011519008011, -204.6249170475634003 ) ) ;
#8382=CARTESIAN_POINT ( 'NONE',  ( -8.872877414587117428, -280.7478352631193275, -198.8399992494221635 ) ) ;
#8383=CARTESIAN_POINT ( 'NONE',  ( -2.395947042261342474, -280.1684228281034166, -201.7567546120976090 ) ) ;
#8385=CARTESIAN_POINT ( 'NONE',  ( 24.38176773647593976, -286.1298346619964263, -312.9890750372579191 ) ) ;
#8387=CARTESIAN_POINT ( 'NONE',  ( -72.69748089556026116, -277.7182422316141128, -205.0860519294942605 ) ) ;
#8388=CARTESIAN_POINT ( 'NONE',  ( -75.75599263695316665, -281.5643120534864465, -334.8367351056810435 ) ) ;
#8389=CARTESIAN_POINT ( 'NONE',  ( 85.24291055932573613, 81.26895824411224112, -298.9807373830735742 ) ) ;
#8390=CARTESIAN_POINT ( 'NONE',  ( -112.1181239977252346, -276.8393319260856629, -285.6308420171541229 ) ) ;
#8392=CARTESIAN_POINT ( 'NONE',  ( -100.7331994143008558, -284.0450582960532415, -227.1047287568084130 ) ) ;
#8393=CARTESIAN_POINT ( 'NONE',  ( -35.15089380731298263, -299.0214930645661298, -197.1254609449464965 ) ) ;
#8394=CARTESIAN_POINT ( 'NONE',  ( -108.6235390214026637, -274.3303832631097521, -242.6925605078068031 ) ) ;
#8395=CARTESIAN_POINT ( 'NONE',  ( 33.91296414719582231, -275.4301550202109752, -286.3823058924789393 ) ) ;
#8396=CARTESIAN_POINT ( 'NONE',  ( -2.184280600849622278, -296.5868824753964077, -336.6103180035956370 ) ) ;
#8397=CARTESIAN_POINT ( 'NONE',  ( -37.49945962628935803, -289.2207188155298923, -347.3740282608129064 ) ) ;
#8398=CARTESIAN_POINT ( 'NONE',  ( 35.94075556086367840, -279.3972474518482727, -251.9492769681368998 ) ) ;
#8399=CARTESIAN_POINT ( 'NONE',  ( 33.32523746210740967, -292.9957822347540173, -239.7803407506089002 ) ) ;
#8400=CARTESIAN_POINT ( 'NONE',  ( -92.59712090189616163, -288.9271287212538368, -318.5019460893274186 ) ) ;
#8401=CARTESIAN_POINT ( 'NONE',  ( 21.55379671925705054, -290.9141717075581823, -223.9043814857781740 ) ) ;
#8402=VERTEX_POINT ( 'NONE', #5148 ) ;
#8404=CARTESIAN_POINT ( 'NONE',  ( -92.59893437561237306, -290.7403210453661018, -222.5633512448363547 ) ) ;
#8406=CARTESIAN_POINT ( 'NONE',  ( -1.091284337424976991, -287.4625440613063461, -202.6948223219712304 ) ) ;
#8407=CARTESIAN_POINT ( 'NONE',  ( 7.450504543161046378, -296.9090924074130839, -326.4764044574609443 ) ) ;
#8408=CARTESIAN_POINT ( 'NONE',  ( 26.30992240531349680, -293.1780110962217805, -313.2713867045764573 ) ) ;
#8409=CARTESIAN_POINT ( 'NONE',  ( -31.65611837700087250, -284.2969967563731188, -346.6695985675668226 ) ) ;
#8410=CARTESIAN_POINT ( 'NONE',  ( -109.8729977947918286, -284.2707679874577025, -279.0562481778311508 ) ) ;
#8411=CARTESIAN_POINT ( 'NONE',  ( 25.80781410736804560, -277.3807122431420566, -307.9560954270891671 ) ) ;
#8412=CARTESIAN_POINT ( 'NONE',  ( 37.28529766639027088, -291.6138401943479153, -273.5845930215531894 ) ) ;
#8413=CARTESIAN_POINT ( 'NONE',  ( -68.43690893236576755, -272.4292298983943965, -203.8626229172665774 ) ) ;
#8415=CARTESIAN_POINT ( 'NONE',  ( -104.9628119525177112, -256.0684274861638983, -326.9234398911233939 ) ) ;
#8416=CARTESIAN_POINT ( 'NONE',  ( 24.00955426602381948, -293.8384824104831523, -316.8559335633037790 ) ) ;
#8417=CARTESIAN_POINT ( 'NONE',  ( 20.62134535090654452, -288.8244461877017670, -223.6333331477684396 ) ) ;
#8418=CARTESIAN_POINT ( 'NONE',  ( -110.0482693383470263, -297.3233503965265641, -294.7588085118717345 ) ) ;
#8419=CARTESIAN_POINT ( 'NONE',  ( 31.06705521557221417, -287.8584378253083287, -244.4474542360500777 ) ) ;
#8420=CARTESIAN_POINT ( 'NONE',  ( -104.5816995602165065, -278.0920755391292118, -233.3259632141318036 ) ) ;
#8421=CARTESIAN_POINT ( 'NONE',  ( -70.75606971522442734, -296.1326914751398931, -339.6344899498650989 ) ) ;
#8422=CARTESIAN_POINT ( 'NONE',  ( 7.189072363802494259, -286.5926370044257396, -331.7227481071446391 ) ) ;
#8423=CARTESIAN_POINT ( 'NONE',  ( -16.50852077234483062, -295.1235046919684919, -344.5224964348305434 ) ) ;
#8424=CARTESIAN_POINT ( 'NONE',  ( -25.40981683922824885, -292.5415750500928311, -198.2699299406296518 ) ) ;
#8426=DIRECTION ( 'NONE',  ( 1.000000000000000000, 0.000000000000000000, 0.000000000000000000 ) ) ;
#8427=CARTESIAN_POINT ( 'NONE',  ( -107.1748277085172987, -264.8307257489187236, -305.4825756969687518 ) ) ;
#8428=CARTESIAN_POINT ( 'NONE',  ( 36.01922953829974006, -288.8045206300831182, -249.1764845995975577 ) ) ;
#8429=CARTESIAN_POINT ( 'NONE',  ( -111.2869819898779866, -281.6237833571633473, -305.9350535429201159 ) ) ;
#8431=CARTESIAN_POINT ( 'NONE',  ( -67.31506793197156924, -279.0178491600407824, -199.5450886581959935 ) ) ;
#8432=CARTESIAN_POINT ( 'NONE',  ( 19.33683420826664090, -282.8732092295673510, -221.4786666618553852 ) ) ;
#8433=CARTESIAN_POINT ( 'NONE',  ( 191.3098834081771997, 269.0209914007751308, -138.7723537854704148 ) ) ;
#8434=CARTESIAN_POINT ( 'NONE',  ( -93.47445018655095339, -283.8389138508416067, -218.4403628813092837 ) ) ;
#8435=CARTESIAN_POINT ( 'NONE',  ( 35.41296738518497023, -285.8364764181033593, -286.1711271937955416 ) ) ;
#8436=CARTESIAN_POINT ( 'NONE',  ( -31.38124961174612437, -275.9870526523563967, -194.8180655509988242 ) ) ;
#8437=CARTESIAN_POINT ( 'NONE',  ( -108.2361819950270387, -297.2779933882924297, -252.6474665598731235 ) ) ;
#8438=CARTESIAN_POINT ( 'NONE',  ( 28.83134217002636746, -292.6681936955410492, -302.4529762751967610 ) ) ;
#8439=CARTESIAN_POINT ( 'NONE',  ( -109.5134036462223435, -279.5412097394954003, -243.6638293505802721 ) ) ;
#8440=CARTESIAN_POINT ( 'NONE',  ( 31.26176204935996594, -275.8863599465067864, -295.4592619193037422 ) ) ;
#8441=CARTESIAN_POINT ( 'NONE',  ( -67.42709771540076247, -274.7463377502214144, -199.8177883026089035 ) ) ;
#8442=CARTESIAN_POINT ( 'NONE',  ( -68.90078820814900951, -276.3777754378377267, -340.2719358146214859 ) ) ;
#8444=CARTESIAN_POINT ( 'NONE',  ( -43.31028530026550527, -275.1272398593608273, -345.1739368166437885 ) ) ;
#8445=CARTESIAN_POINT ( 'NONE',  ( -113.6442382214117117, -297.9149350527327442, -275.3193654817033007 ) ) ;
#8446=CARTESIAN_POINT ( 'NONE',  ( -95.99890600148557951, -275.6948066931273615, -223.6242672951989618 ) ) ;
#8447=CARTESIAN_POINT ( 'NONE',  ( 168.8235619055982113, 230.3815547064285738, -190.2228674158758395 ) ) ;
#8448=CARTESIAN_POINT ( 'NONE',  ( -96.02159608354469356, -286.2460113764979610, -226.4191575681084885 ) ) ;
#8449=CARTESIAN_POINT ( 'NONE',  ( -92.67802161734913113, -285.5918050138986928, -322.4557623740048484 ) ) ;
#8450=CARTESIAN_POINT ( 'NONE',  ( -25.11661920508774415, -285.5606085391307261, -198.2372836293438354 ) ) ;
#8451=CARTESIAN_POINT ( 'NONE',  ( -95.40780278049497554, -277.5875278856383375, -224.7911629146941266 ) ) ;
#8452=CARTESIAN_POINT ( 'NONE',  ( -109.2845303047393770, -286.1749746913413901, -288.6667091822764633 ) ) ;
#8453=CARTESIAN_POINT ( 'NONE',  ( -108.9589396283162728, -277.2590362881911119, -252.9922158627122428 ) ) ;
#8454=CARTESIAN_POINT ( 'NONE',  ( -54.01091033362814642, -278.3507675604900555, -341.8022966407779109 ) ) ;
#8456=CARTESIAN_POINT ( 'NONE',  ( -110.2506496594334919, -273.1162838474767227, -264.9151045739267261 ) ) ;
#8458=CARTESIAN_POINT ( 'NONE',  ( 38.63349031472916550, -282.2067100469844831, -258.5302816038997094 ) ) ;
#8459=CARTESIAN_POINT ( 'NONE',  ( 39.12088293316512022, -281.9317231116910989, -261.3509419643702358 ) ) ;
#8463=CARTESIAN_POINT ( 'NONE',  ( 30.30808499766753883, -288.9664049285214560, -236.2464283276986237 ) ) ;
#8464=CARTESIAN_POINT ( 'NONE',  ( -106.0778620103985901, -288.8014437903967178, -304.0768052511444921 ) ) ;
#8465=CARTESIAN_POINT ( 'NONE',  ( -71.73188240598024379, -296.7826183578704331, -205.7719944301186956 ) ) ;
#8466=CARTESIAN_POINT ( 'NONE',  ( 21.23819028622834537, -292.2280225474484610, -220.5242421328150328 ) ) ;
#8467=CARTESIAN_POINT ( 'NONE',  ( 34.67767361159377515, -285.8279410744211759, -254.7432576713999310 ) ) ;
#8468=CARTESIAN_POINT ( 'NONE',  ( 1.608192231784646431, -287.0949351505607297, -332.7973318479549789 ) ) ;
#8469=CARTESIAN_POINT ( 'NONE',  ( -14.45668811898826789, -287.5604909296918663, -200.5696858399135465 ) ) ;
#8470=CARTESIAN_POINT ( 'NONE',  ( -112.3841908609287543, -276.5367145900733021, -271.5505799756937790 ) ) ;
#8471=CARTESIAN_POINT ( 'NONE',  ( 37.63997241300206298, -289.5310266062551250, -268.7029778690200601 ) ) ;
#8472=CARTESIAN_POINT ( 'NONE',  ( -106.0657691578680470, -288.1525095454317693, -300.9364141708742295 ) ) ;
#8473=CARTESIAN_POINT ( 'NONE',  ( -91.83212262548094884, -284.7951455964642946, -319.3105709106018821 ) ) ;
#8474=CARTESIAN_POINT ( 'NONE',  ( -102.2032465073414897, -292.0446285120938796, -308.4509585775351184 ) ) ;
#8478=CARTESIAN_POINT ( 'NONE',  ( -63.02080052824070577, -275.6992839420630048, -199.5162832753156863 ) ) ;
#8479=CARTESIAN_POINT ( 'NONE',  ( -11.67694546944097311, -279.5921199740473639, -201.7953349648843187 ) ) ;
#8480=CARTESIAN_POINT ( 'NONE',  ( 4.485042898639600040, -280.4881251836865772, -332.6776331543525771 ) ) ;
#8481=CARTESIAN_POINT ( 'NONE',  ( -39.11438272366691393, -294.2710400302972289, -347.1791914907149703 ) ) ;
#8482=CARTESIAN_POINT ( 'NONE',  ( -89.94686466845699613, -271.5363821796510138, -218.2970163721493293 ) ) ;
#8483=CARTESIAN_POINT ( 'NONE',  ( -21.36738178200117133, -274.9256816697155728, -343.1199456173536646 ) ) ;
#8484=CARTESIAN_POINT ( 'NONE',  ( -109.7646638889822128, -298.0310712164553024, -257.8648065737219213 ) ) ;
#8486=CARTESIAN_POINT ( 'NONE',  ( -102.2616301707950157, -294.2695249540354894, -309.8500619489861947 ) ) ;
#8487=CARTESIAN_POINT ( 'NONE',  ( 36.23181522101855023, -295.0184566641829633, -273.4961155717368797 ) ) ;
#8488=FACE_OUTER_BOUND ( 'NONE', #40766, .T. ) ;
#8489=CARTESIAN_POINT ( 'NONE',  ( -18.16836128501384806, -295.6014577201963789, -340.9655428019839292 ) ) ;
#8491=CARTESIAN_POINT ( 'NONE',  ( -40.71700741363184051, -284.0301395286036268, -195.0304658060662462 ) ) ;
#8492=CARTESIAN_POINT ( 'NONE',  ( -96.88273702143361277, -297.1419161421789568, -228.1252928377322746 ) ) ;
#8493=CARTESIAN_POINT ( 'NONE',  ( -79.15972554674409878, -283.5997481412384218, -335.0159921227520385 ) ) ;
#8494=CARTESIAN_POINT ( 'NONE',  ( -21.99413509095603558, -284.7771447667798839, -344.3460248394388259 ) ) ;
#8495=CARTESIAN_POINT ( 'NONE',  ( 21.47012229830211893, -287.8882004341004404, -320.0291543288612957 ) ) ;
#8496=CARTESIAN_POINT ( 'NONE',  ( 34.39366436981235609, -291.2748186313027645, -248.8735217326230611 ) ) ;
#8497=CARTESIAN_POINT ( 'NONE',  ( -113.9782757722468745, -277.8136749155742677, -277.3135967240182822 ) ) ;
#8498=CARTESIAN_POINT ( 'NONE',  ( -85.33152481854862970, -275.1952119285918457, -330.4860931364851808 ) ) ;
#8500=CARTESIAN_POINT ( 'NONE',  ( 18.08607435315859036, -285.6649154893116815, -222.2477900817396517 ) ) ;
#8501=CARTESIAN_POINT ( 'NONE',  ( -108.0767089125435660, -289.8509105964187711, -240.7291919360389727 ) ) ;
#8503=CARTESIAN_POINT ( 'NONE',  ( -110.0999810773095788, -279.6797307292029586, -293.8731295310336691 ) ) ;
#8504=CARTESIAN_POINT ( 'NONE',  ( -63.71466804734471623, -293.4143918343031032, -340.9505886250406661 ) ) ;
#8505=CARTESIAN_POINT ( 'NONE',  ( 35.54122530967838145, -281.1596458456153300, -265.8703868246133766 ) ) ;
#8506=CARTESIAN_POINT ( 'NONE',  ( -61.58955177424697069, -295.5252286361533720, -343.4992870877245537 ) ) ;
#8507=CARTESIAN_POINT ( 'NONE',  ( 28.88151341569323804, -285.1505904973551537, -233.8684258384276404 ) ) ;
#8508=CARTESIAN_POINT ( 'NONE',  ( -98.62973332764182999, -281.1395390396712060, -227.1317571657514804 ) ) ;
#8509=CARTESIAN_POINT ( 'NONE',  ( -10.41460458241496490, -293.7506915505009033, -338.4664773442113983 ) ) ;
#8510=CARTESIAN_POINT ( 'NONE',  ( -33.43817532355726740, -296.1008595978869380, -195.3624401095650853 ) ) ;
#8513=CARTESIAN_POINT ( 'NONE',  ( 30.82662058890845103, -283.9340214632740640, -300.9007367978998104 ) ) ;
#8514=CARTESIAN_POINT ( 'NONE',  ( -107.6637421984649166, -295.7980334214305458, -290.1802713656869059 ) ) ;
#8516=CARTESIAN_POINT ( 'NONE',  ( -110.4683760289727132, -275.8380690714489560, -287.0191576251351080 ) ) ;
#8517=CARTESIAN_POINT ( 'NONE',  ( -15.81278041597468409, -273.5207998835425656, -196.5450327971991840 ) ) ;
#8518=CARTESIAN_POINT ( 'NONE',  ( -102.8463662289646692, -289.9488796982461736, -302.5812781853688875 ) ) ;
#8519=CARTESIAN_POINT ( 'NONE',  ( -109.2878386642281470, -280.2814157945992406, -254.3514499904401873 ) ) ;
#8520=CARTESIAN_POINT ( 'NONE',  ( -72.30452460671274650, -275.1819656868574384, -205.3115447985777848 ) ) ;
#8521=CARTESIAN_POINT ( 'NONE',  ( 19.20369637442949440, -283.8538039479970507, -321.5172843107293374 ) ) ;
#8522=CARTESIAN_POINT ( 'NONE',  ( -14.16904126558389621, -279.1542827669932763, -200.6643054074703514 ) ) ;
#8523=CARTESIAN_POINT ( 'NONE',  ( -71.33719196742354995, -279.5012423309570408, -337.2139951600037762 ) ) ;
#8525=CARTESIAN_POINT ( 'NONE',  ( -36.93760085196832677, -273.8904336506888058, -193.3491261987479390 ) ) ;
#8526=CARTESIAN_POINT ( 'NONE',  ( -94.56212658089165757, -293.1349209898801860, -222.7267480702109310 ) ) ;
#8527=DIRECTION ( 'NONE',  ( -0.000000000000000000, 0.000000000000000000, 1.000000000000000000 ) ) ;
#8528=CARTESIAN_POINT ( 'NONE',  ( 129.8975571001389540, -299.5541904835127980, -195.3611179825600175 ) ) ;
#8529=CARTESIAN_POINT ( 'NONE',  ( 38.00600409903060495, -291.7987623753188586, -278.7815107990267620 ) ) ;
#8530=CARTESIAN_POINT ( 'NONE',  ( -5.275392787371918857, -273.9935598726879675, -204.6986685928319787 ) ) ;
#8532=CARTESIAN_POINT ( 'NONE',  ( 34.79080259566576672, -294.7538256067413727, -245.3093311926543265 ) ) ;
#8533=CARTESIAN_POINT ( 'NONE',  ( -110.4542110544635705, -280.8376638359844719, -287.0812184334320705 ) ) ;
#8534=CARTESIAN_POINT ( 'NONE',  ( -36.39875151458510061, -293.2687978539395885, -193.7510280396973030 ) ) ;
#8535=CARTESIAN_POINT ( 'NONE',  ( 34.01424054599034719, -289.2602468523275547, -247.7714660062942187 ) ) ;
#8536=CARTESIAN_POINT ( 'NONE',  ( 36.84118362251066969, -273.4252965534334407, -260.5159067252370733 ) ) ;
#8537=CARTESIAN_POINT ( 'NONE',  ( 12.73412476348975986, -278.2678016501989191, -325.5103546945414337 ) ) ;
#8538=CARTESIAN_POINT ( 'NONE',  ( 21.64969254740626425, -292.2588737147723918, -315.7838498414823221 ) ) ;
#8539=CARTESIAN_POINT ( 'NONE',  ( -17.34123119427936999, -282.1680077757955019, -197.2838525683130513 ) ) ;
#8541=CARTESIAN_POINT ( 'NONE',  ( -32.14843171769513219, -282.6515559556271455, -343.1973551863935654 ) ) ;
#8542=CARTESIAN_POINT ( 'NONE',  ( -100.0043843694782169, -280.2191986184222401, -226.1470872486226824 ) ) ;
#8543=CARTESIAN_POINT ( 'NONE',  ( -13.55985214278771167, -281.5450195675607574, -343.1789209173725226 ) ) ;
#8544=CARTESIAN_POINT ( 'NONE',  ( 19.71038571434487707, -277.1928535865182539, -321.7410865202629680 ) ) ;
#8545=CARTESIAN_POINT ( 'NONE',  ( 19.37495490397807174, -277.7716300887892658, -321.4289768659267565 ) ) ;
#8546=CARTESIAN_POINT ( 'NONE',  ( 17.40634833298267736, -284.6948066931273047, -313.9805196606274080 ) ) ;
#8549=CARTESIAN_POINT ( 'NONE',  ( -35.78852967049083844, -300.0717513479477816, -195.3605797401941118 ) ) ;
#8550=CARTESIAN_POINT ( 'NONE',  ( -107.6958101301144950, -291.9037945579524376, -249.7125039511552416 ) ) ;
#8551=CARTESIAN_POINT ( 'NONE',  ( -111.9953503259433347, -276.6049358226782715, -267.8278428600737584 ) ) ;
#8552=CARTESIAN_POINT ( 'NONE',  ( -96.48701543572346395, -291.6639952600055494, -318.0870361192027076 ) ) ;
#8553=CARTESIAN_POINT ( 'NONE',  ( 12.97932452968493244, -292.1263441446682236, -217.3357736142462784 ) ) ;
#8554=CARTESIAN_POINT ( 'NONE',  ( 39.28559346629512561, -287.1463276615442624, -277.2737715623856616 ) ) ;
#8556=CARTESIAN_POINT ( 'NONE',  ( -108.7982112931249219, -283.1929420817123173, -251.9109844030388956 ) ) ;
#8557=CARTESIAN_POINT ( 'NONE',  ( -111.4807276213506952, -292.4732866331131618, -265.6809624300449855 ) ) ;
#8558=CARTESIAN_POINT ( 'NONE',  ( -110.1026317070394214, -283.1857713856381338, -258.5956585211296215 ) ) ;
#8559=CARTESIAN_POINT ( 'NONE',  ( -32.95016836994529541, -281.4238135536698451, -196.9992891652491380 ) ) ;
#8561=CARTESIAN_POINT ( 'NONE',  ( -100.4802292629586873, -290.9150069585285792, -314.0228443770856188 ) ) ;
#8562=CARTESIAN_POINT ( 'NONE',  ( 34.12407828448477431, -281.8435774252426427, -255.1149938951859326 ) ) ;
#8563=CARTESIAN_POINT ( 'NONE',  ( -36.36792057564785097, -290.8590369371053157, -193.7514131717549901 ) ) ;
#8564=CARTESIAN_POINT ( 'NONE',  ( 39.18753752156337811, -288.4412987802419366, -277.2483964668076055 ) ) ;
#8565=CARTESIAN_POINT ( 'NONE',  ( 33.80012921578681073, -287.6703157568388178, -240.9240623464333737 ) ) ;
#8566=CARTESIAN_POINT ( 'NONE',  ( -81.48026296028501747, -285.5989772554643196, -212.2165801858669170 ) ) ;
#8569=CARTESIAN_POINT ( 'NONE',  ( -27.87824375417724809, -296.7937706180347845, -345.5850169843606068 ) ) ;
#8570=CARTESIAN_POINT ( 'NONE',  ( -86.09403039252175915, -294.3968788215267978, -329.3230426901273518 ) ) ;
#8571=CARTESIAN_POINT ( 'NONE',  ( -27.00009642510053354, -275.9761725206695928, -342.8625640407503283 ) ) ;
#8573=CARTESIAN_POINT ( 'NONE',  ( -20.52926933915206220, -297.6060565333928594, -193.4648508431261007 ) ) ;
#8574=CARTESIAN_POINT ( 'NONE',  ( 35.16882939122410789, -291.8592658757383447, -257.1405311304141605 ) ) ;
#8575=CARTESIAN_POINT ( 'NONE',  ( -110.1428868112222403, -294.6175229179860935, -283.7716515658402727 ) ) ;
#8576=CARTESIAN_POINT ( 'NONE',  ( 9.088221398714868116, -293.9108085946446636, -213.4498648993220513 ) ) ;
#8577=CARTESIAN_POINT ( 'NONE',  ( 18.70406148533283996, -293.9632502869982318, -223.1054444647598700 ) ) ;
#8579=CARTESIAN_POINT ( 'NONE',  ( 22.55234686636103802, -292.1718727129482431, -315.7784226645349577 ) ) ;
#8580=CARTESIAN_POINT ( 'NONE',  ( -60.29593098400137308, -299.7548470042601707, -198.9062182013545907 ) ) ;
#8581=CARTESIAN_POINT ( 'NONE',  ( -58.74648930122697976, -290.2770122978339487, -340.4515322190196684 ) ) ;
#8582=CARTESIAN_POINT ( 'NONE',  ( -3.130094142473434538, -294.9202725909191827, -334.8719969311759996 ) ) ;
#8583=CARTESIAN_POINT ( 'NONE',  ( -83.83139389325179991, -279.6663365261928220, -329.7326753621404123 ) ) ;
#8584=CARTESIAN_POINT ( 'NONE',  ( -31.09719897742591854, -278.8141786934916126, -194.0571780743866555 ) ) ;
#8586=CARTESIAN_POINT ( 'NONE',  ( -110.0028304246662429, -272.2185276980334265, -245.1882569914864689 ) ) ;
#8587=CARTESIAN_POINT ( 'NONE',  ( 28.10978045569169126, -280.1064891649999140, -305.8212065982333456 ) ) ;
#8588=CARTESIAN_POINT ( 'NONE',  ( -113.4342314520543908, -276.9008974433064623, -274.4067440580694210 ) ) ;
#8589=CARTESIAN_POINT ( 'NONE',  ( -106.8084080859245404, -276.9258367053010943, -241.6486658152932421 ) ) ;
#8591=CARTESIAN_POINT ( 'NONE',  ( -41.88219090209978646, -296.6785613736013829, -197.0083578293589994 ) ) ;
#8594=CARTESIAN_POINT ( 'NONE',  ( -94.39865646931430376, -289.2516887158759573, -221.1183341442224446 ) ) ;
#8595=CARTESIAN_POINT ( 'NONE',  ( -113.1720195082019842, -290.7193651635979563, -256.9909024753625317 ) ) ;
#8596=CARTESIAN_POINT ( 'NONE',  ( -27.26805092027870714, -276.1799215185916410, -195.8203715622629772 ) ) ;
#8597=CARTESIAN_POINT ( 'NONE',  ( -66.25819306634969053, -295.6725654145596991, -201.3403612176760191 ) ) ;
#8598=CARTESIAN_POINT ( 'NONE',  ( -24.57050823684281937, -282.0904470567856492, -346.1848723641564902 ) ) ;
#8600=CARTESIAN_POINT ( 'NONE',  ( 30.08590757004203908, -279.9861861303398882, -303.3190077482742595 ) ) ;
#8602=CARTESIAN_POINT ( 'NONE',  ( -52.43652374490492463, -290.6495580378345380, -198.4808312817270064 ) ) ;
#8603=CARTESIAN_POINT ( 'NONE',  ( -55.02804012543816725, -283.9620341050729166, -198.2103743442108907 ) ) ;
#8604=CARTESIAN_POINT ( 'NONE',  ( 104.1964229570258311, -299.5541904835127980, -193.4651424135224147 ) ) ;
#8606=FACE_BOUND ( 'NONE', #32045, .T. ) ;
#8607=CARTESIAN_POINT ( 'NONE',  ( 20.02231082032096054, -290.8839164988875154, -222.0457901881875387 ) ) ;
#8608=CARTESIAN_POINT ( 'NONE',  ( -74.39753248658713858, -279.1539399645397452, -334.1835725237709198 ) ) ;
#8609=CARTESIAN_POINT ( 'NONE',  ( -99.45744512396487380, -285.1587094193211556, -315.2787817480978561 ) ) ;
#8610=CARTESIAN_POINT ( 'NONE',  ( -18.87773257458828269, -272.3677574155432239, -197.0377734563224124 ) ) ;
#8611=CARTESIAN_POINT ( 'NONE',  ( -25.14182038879835090, -286.2119169001420005, -198.3364711641547729 ) ) ;
#8612=CARTESIAN_POINT ( 'NONE',  ( 36.19168952555523333, -277.0293220700342545, -274.3264308221850456 ) ) ;
#8613=CARTESIAN_POINT ( 'NONE',  ( -53.98073997701444426, -278.0739732817420986, -341.6576290220816645 ) ) ;
#8614=CARTESIAN_POINT ( 'NONE',  ( -92.90001816390980593, -285.8494174581897482, -320.7614435924210170 ) ) ;
#8617=CARTESIAN_POINT ( 'NONE',  ( -110.8004322634721035, -296.0949207064991811, -293.4880331806546110 ) ) ;
#8618=CARTESIAN_POINT ( 'NONE',  ( -14.07677004862288861, -288.3351825727351638, -199.3802610569312606 ) ) ;
#8620=CARTESIAN_POINT ( 'NONE',  ( -37.30987171927208834, -295.5523547857347353, -190.3611179825600175 ) ) ;
#8621=CARTESIAN_POINT ( 'NONE',  ( -45.22785470368222605, -278.8749529551315618, -194.0239970231942550 ) ) ;
#8622=CARTESIAN_POINT ( 'NONE',  ( -73.04069625457167092, -289.9870104868959402, -203.0260799935663556 ) ) ;
#8623=CARTESIAN_POINT ( 'NONE',  ( -109.6561591126852591, -285.8868621229585187, -284.5500846738510177 ) ) ;
#8624=CARTESIAN_POINT ( 'NONE',  ( -75.04098038060307374, -281.3031154322780480, -206.6096716857336730 ) ) ;
#8625=CARTESIAN_POINT ( 'NONE',  ( 29.85324596469640568, -289.4528955526334357, -306.8510135246826849 ) ) ;
#8626=CARTESIAN_POINT ( 'NONE',  ( 37.01219629029702674, -283.4212380202898771, -260.1525991322405957 ) ) ;
#8627=CARTESIAN_POINT ( 'NONE',  ( -7.882673134869967235, -276.8433798928666079, -341.5172732836531395 ) ) ;
#8628=CARTESIAN_POINT ( 'NONE',  ( -98.20968232412593579, -295.1623437260620335, -227.1530684139967491 ) ) ;
#8629=CARTESIAN_POINT ( 'NONE',  ( -86.80309730374099786, -279.2196916953470804, -211.2783179846476571 ) ) ;
#8630=CARTESIAN_POINT ( 'NONE',  ( -58.33382395624661143, -299.6988598215668844, -198.9423184080384601 ) ) ;
#8632=CARTESIAN_POINT ( 'NONE',  ( -54.49178911615187815, -294.3376638359846424, -195.3683826091709363 ) ) ;
#8633=CARTESIAN_POINT ( 'NONE',  ( -21.54330697732822131, -272.4918891999190009, -196.0349127440500752 ) ) ;
#8635=CARTESIAN_POINT ( 'NONE',  ( -108.0305307688355470, -278.3040167540164020, -251.8437045672945942 ) ) ;
#8636=CARTESIAN_POINT ( 'NONE',  ( 34.83205540677287360, -277.0846484153361189, -296.1877306781838683 ) ) ;
#8637=CARTESIAN_POINT ( 'NONE',  ( -74.17366008294015955, -282.5877494812569921, -337.7719499203433884 ) ) ;
#8638=CARTESIAN_POINT ( 'NONE',  ( -18.18997404698201947, -290.5622206765494298, -341.9069929114824617 ) ) ;
#8639=CARTESIAN_POINT ( 'NONE',  ( -3.809375465612989231, -299.9848854821569262, -194.0459541100681236 ) ) ;
#8640=CARTESIAN_POINT ( 'NONE',  ( -108.5253362119391483, -298.1196808925650998, -241.9183460448227834 ) ) ;
#8641=CARTESIAN_POINT ( 'NONE',  ( -39.72247161212852973, -297.0822525065316881, -345.1693177223515931 ) ) ;
#8642=CARTESIAN_POINT ( 'NONE',  ( 34.71812903033746522, -279.8122422826048137, -290.5455042772341017 ) ) ;
#8643=CARTESIAN_POINT ( 'NONE',  ( 8.357346866369255167, -272.7013091175344357, -211.3404105707781468 ) ) ;
#8644=CARTESIAN_POINT ( 'NONE',  ( -105.9675634679459506, -286.5816652309669621, -237.2411648689164565 ) ) ;
#8645=CARTESIAN_POINT ( 'NONE',  ( 3.776662570077772063, -287.4049043132056909, -331.1142189481298033 ) ) ;
#8646=CARTESIAN_POINT ( 'NONE',  ( 162.7515160168861428, 219.2654253216233542, -204.9874331692004432 ) ) ;
#8648=CARTESIAN_POINT ( 'NONE',  ( 36.21224550453401747, -286.3888206581659688, -291.1074510879297463 ) ) ;
#8649=CARTESIAN_POINT ( 'NONE',  ( -63.83252280476894924, -289.0739064444559858, -338.4618027553802904 ) ) ;
#8651=CARTESIAN_POINT ( 'NONE',  ( -78.36875182783701632, -286.5934641132845968, -205.5670323099561188 ) ) ;
#8652=CARTESIAN_POINT ( 'NONE',  ( 22.29564931330443045, -275.2971930838963317, -228.2031003941001757 ) ) ;
#8653=CARTESIAN_POINT ( 'NONE',  ( -7.298571768429359174, -291.3573588888247627, -199.7855107588698615 ) ) ;
#8654=CARTESIAN_POINT ( 'NONE',  ( 38.77155861461756814, -282.3407936067129640, -281.3194312715824594 ) ) ;
#8655=CARTESIAN_POINT ( 'NONE',  ( 38.59024674462135351, -283.1740488553423347, -278.4258361406720610 ) ) ;
#8656=CARTESIAN_POINT ( 'NONE',  ( 11.48246731664224107, -282.7297812828086876, -329.9443407566290034 ) ) ;
#8657=CARTESIAN_POINT ( 'NONE',  ( 34.08498995237063411, -281.6845371941750500, -255.1254107772410009 ) ) ;
#8658=CARTESIAN_POINT ( 'NONE',  ( -20.25526795762938548, -274.3380690714490697, -345.3683826091709648 ) ) ;
#8659=CARTESIAN_POINT ( 'NONE',  ( -95.38918660201169075, -240.2644329508013357, -341.8810175719231097 ) ) ;
#8661=CARTESIAN_POINT ( 'NONE',  ( -26.73715559290007704, -278.9171112223259001, -344.4392663105000452 ) ) ;
#8662=CARTESIAN_POINT ( 'NONE',  ( 4.645253263068006788, -57.92935080797366254, -354.0998759884595302 ) ) ;
#8663=CARTESIAN_POINT ( 'NONE',  ( 101.6986848688134586, 115.4960904796168393, -279.9121412288012039 ) ) ;
#8664=CARTESIAN_POINT ( 'NONE',  ( -110.3135459398219922, -295.9581595143036452, -266.0019452707307437 ) ) ;
#8665=CARTESIAN_POINT ( 'NONE',  ( 36.64671156940783447, -292.7945491653310341, -249.2123443802435929 ) ) ;
#8666=CARTESIAN_POINT ( 'NONE',  ( 26.38539103948928499, -24.50260877297474948, -341.6991638436127232 ) ) ;
#8667=CARTESIAN_POINT ( 'NONE',  ( -99.43208137315983208, -295.7216227387097547, -225.8258415100113723 ) ) ;
#8668=CARTESIAN_POINT ( 'NONE',  ( -76.30824931387375898, -287.9825075597531736, -333.0352630439224413 ) ) ;
#8669=CARTESIAN_POINT ( 'NONE',  ( -53.39376664352313639, -297.1205017808284197, -342.8929181222869715 ) ) ;
#8670=CARTESIAN_POINT ( 'NONE',  ( 8.299210339719618190, -289.7275113414931980, -327.9645099680136013 ) ) ;
#8672=CARTESIAN_POINT ( 'NONE',  ( -34.85023741128619434, -295.9628159430980645, -347.0853829001013082 ) ) ;
#8673=CARTESIAN_POINT ( 'NONE',  ( -74.75700363222532019, -286.0317908867681354, -207.6069666827362425 ) ) ;
#8674=CARTESIAN_POINT ( 'NONE',  ( -98.76481319911852097, -295.9593143616284578, -224.5657682304249363 ) ) ;
#8675=CARTESIAN_POINT ( 'NONE',  ( -37.80433812347801847, -292.8493236978347909, -193.5239864155846305 ) ) ;
#8676=CARTESIAN_POINT ( 'NONE',  ( 37.03868280770084453, -294.2910009028161085, -290.0356074990441471 ) ) ;
#8677=CARTESIAN_POINT ( 'NONE',  ( -109.2771301956596943, -290.8865011739408715, -257.6509473832102799 ) ) ;
#8680=CARTESIAN_POINT ( 'NONE',  ( -38.36294310990003709, -275.9595924577715209, -194.8080156985693066 ) ) ;
#8681=CARTESIAN_POINT ( 'NONE',  ( 32.65071107476301648, -274.7464654801361235, -301.4910246883414402 ) ) ;
#8684=CARTESIAN_POINT ( 'NONE',  ( -65.07874458106763882, -276.9125228242414778, -342.1821386233470434 ) ) ;
#8685=CARTESIAN_POINT ( 'NONE',  ( -43.52910050740107550, -272.3726998332504650, -196.7696826814672306 ) ) ;
#8686=CARTESIAN_POINT ( 'NONE',  ( -46.07656276909249016, -275.3035396841446527, -344.1321212506566667 ) ) ;
#8687=CARTESIAN_POINT ( 'NONE',  ( -54.29631431284116161, -274.9088878367037410, -199.0395424918422691 ) ) ;
#8688=CARTESIAN_POINT ( 'NONE',  ( -93.96792944599680197, -274.1493470417372578, -223.8992986894124897 ) ) ;
#8689=CARTESIAN_POINT ( 'NONE',  ( -100.3805962421122331, -274.8797411425118185, -227.8401535387212675 ) ) ;
#8690=CARTESIAN_POINT ( 'NONE',  ( -84.75339119934942289, -271.4223757795686538, -211.7903202288688931 ) ) ;
#8691=CARTESIAN_POINT ( 'NONE',  ( -66.08558870448167966, -296.0899854878438759, -337.5748185049633321 ) ) ;
#8692=CARTESIAN_POINT ( 'NONE',  ( 24.91614604700444957, -292.6656620354552842, -309.6911681145660395 ) ) ;
#8694=CARTESIAN_POINT ( 'NONE',  ( -68.98433154738133055, -277.9495398045638694, -340.5058945935911652 ) ) ;
#8695=CARTESIAN_POINT ( 'NONE',  ( 35.64286128180913948, -275.6990291148887309, -268.8598517539333557 ) ) ;
#8696=CARTESIAN_POINT ( 'NONE',  ( -110.2209199239085251, -282.9419378392214526, -293.6834746463918009 ) ) ;
#8697=CARTESIAN_POINT ( 'NONE',  ( -105.4931686752748305, -298.1365789482953232, -302.0692519284278319 ) ) ;
#8699=CARTESIAN_POINT ( 'NONE',  ( -42.67572212288514777, -285.1803338228510825, -197.3816916267900865 ) ) ;
#8702=CARTESIAN_POINT ( 'NONE',  ( -110.9718130055678103, -276.8962461782848550, -262.3493589867784408 ) ) ;
#8703=CARTESIAN_POINT ( 'NONE',  ( -45.99525885316750617, -275.7386132035457535, -343.4908149029940319 ) ) ;
#8704=CARTESIAN_POINT ( 'NONE',  ( -111.2793011175721034, -286.7147948671331505, -257.7066023417874021 ) ) ;
#8705=CARTESIAN_POINT ( 'NONE',  ( -21.86518396271576137, -275.4600181604830027, -198.6142856413370623 ) ) ;
#8707=CARTESIAN_POINT ( 'NONE',  ( 38.52290734758198454, -273.8549722713872825, -262.6814432798924486 ) ) ;
#8708=CARTESIAN_POINT ( 'NONE',  ( -97.13388025945299376, -281.1745431911787136, -224.7888128637086709 ) ) ;
#8710=CARTESIAN_POINT ( 'NONE',  ( -65.36643516044743762, -287.6088473957584597, -200.1765167969331003 ) ) ;
#8712=CARTESIAN_POINT ( 'NONE',  ( -73.02013669791863038, -289.5792140193086652, -204.3766296577742025 ) ) ;
#8713=CARTESIAN_POINT ( 'NONE',  ( 82.14177983934591509, -300.1103622902044208, -197.2983025311162066 ) ) ;
#8714=CARTESIAN_POINT ( 'NONE',  ( -91.47451648554300618, -271.9458055172195827, -220.6345298867763631 ) ) ;
#8715=CARTESIAN_POINT ( 'NONE',  ( -84.59740556197802164, -289.5326553064027166, -213.1093600932679806 ) ) ;
#8716=CARTESIAN_POINT ( 'NONE',  ( -112.8392349625790274, -266.9846182459017427, -270.2902299390011081 ) ) ;
#8718=CARTESIAN_POINT ( 'NONE',  ( -4.647837540224855957, -287.1091599749095167, -339.3234098850159057 ) ) ;
#8719=CARTESIAN_POINT ( 'NONE',  ( -100.1461425751381142, -283.3646982768908629, -227.4946649935920391 ) ) ;
#8720=CARTESIAN_POINT ( 'NONE',  ( -105.7106420440656933, -290.8952156425477256, -244.6308149921879078 ) ) ;
#8721=CARTESIAN_POINT ( 'NONE',  ( 22.58284863146822019, -282.3855036991515135, -227.6478486870835525 ) ) ;
#8723=CARTESIAN_POINT ( 'NONE',  ( 34.49083719769880929, -282.1714070554660907, -256.4139442942782239 ) ) ;
#8724=CARTESIAN_POINT ( 'NONE',  ( -90.42165271232587997, -291.7784773398208813, -323.9221152937140573 ) ) ;
#8725=CARTESIAN_POINT ( 'NONE',  ( -34.76156588297511263, -298.2502992953101284, -193.3610472403868243 ) ) ;
#8727=CARTESIAN_POINT ( 'NONE',  ( -79.75296315849625728, -287.7000329597065047, -332.9591212113024881 ) ) ;
#8728=CARTESIAN_POINT ( 'NONE',  ( -1.301494443111259391, -274.5168195144583478, -202.3162535607312691 ) ) ;
#8729=CARTESIAN_POINT ( 'NONE',  ( -34.82655734279133952, -294.0638002857967876, -195.7586993748782902 ) ) ;
#8731=CARTESIAN_POINT ( 'NONE',  ( -20.25526795762937127, -276.7662352645559167, -195.3538533559490702 ) ) ;
#8732=CARTESIAN_POINT ( 'NONE',  ( -51.12670898422591392, -281.9167209665001224, -342.6018041981239435 ) ) ;
#8733=CARTESIAN_POINT ( 'NONE',  ( -112.3791529965137101, -276.6084302471541605, -265.9555429921563814 ) ) ;
#8735=CARTESIAN_POINT ( 'NONE',  ( -36.17886483558234545, -296.4663592219857264, -194.1614229672849206 ) ) ;
#8736=CARTESIAN_POINT ( 'NONE',  ( 20.91313319842510410, -275.5204868133725427, -314.5229460991500900 ) ) ;
#8737=CARTESIAN_POINT ( 'NONE',  ( 19.87194822981332010, -294.4210761875629032, -223.8943565759877004 ) ) ;
#8738=CARTESIAN_POINT ( 'NONE',  ( -62.89401960208366660, -292.6523717872654515, -201.7281272448653908 ) ) ;
#8739=CARTESIAN_POINT ( 'NONE',  ( -95.77064682945967888, -286.9438338828415453, -224.9089101291104100 ) ) ;
#8740=CARTESIAN_POINT ( 'NONE',  ( 39.01871031866595274, -295.0123809232335361, -273.1349254321697231 ) ) ;
#8741=CARTESIAN_POINT ( 'NONE',  ( 38.12264967627783108, -295.0267536753127615, -283.0275053719837501 ) ) ;
#8742=CARTESIAN_POINT ( 'NONE',  ( -58.41026653058792562, -295.1655507889832393, -340.2547193651718658 ) ) ;
#8743=CARTESIAN_POINT ( 'NONE',  ( 37.54808777759830463, -289.4890081764498859, -265.4305154974574066 ) ) ;
#8744=CARTESIAN_POINT ( 'NONE',  ( -113.5990700524482548, -284.5807002303261584, -281.4059909135083331 ) ) ;
#8745=CARTESIAN_POINT ( 'NONE',  ( -43.15412129400511532, -296.0592921269231965, -194.9727899944366527 ) ) ;
#8746=CARTESIAN_POINT ( 'NONE',  ( -102.9191899554285925, -283.8580215166877565, -310.7169457208166818 ) ) ;
#8747=CARTESIAN_POINT ( 'NONE',  ( -98.21270316857264504, -279.9417691240291219, -313.5871004770190780 ) ) ;
#8748=CARTESIAN_POINT ( 'NONE',  ( -87.95729433502280870, -284.1198129014680944, -217.2085815685039165 ) ) ;
#8749=CARTESIAN_POINT ( 'NONE',  ( 36.69635282843014323, -285.7097769775011784, -282.6498183180680144 ) ) ;
#8750=CARTESIAN_POINT ( 'NONE',  ( -76.82821360252853538, -277.6693978044604023, -205.6388062164121493 ) ) ;
#8751=CARTESIAN_POINT ( 'NONE',  ( -107.3349855510151656, -256.5393008024622077, -313.9713749062190686 ) ) ;
#8752=CARTESIAN_POINT ( 'NONE',  ( -95.00176195320742067, -284.6917100414731294, -225.4709301275851487 ) ) ;
#8753=CARTESIAN_POINT ( 'NONE',  ( 28.93531533436184944, -282.2551111191983750, -231.9506254171920716 ) ) ;
#8754=CARTESIAN_POINT ( 'NONE',  ( 0.5925549777742314950, -287.6184451414697492, -337.1580722811984288 ) ) ;
#8755=CARTESIAN_POINT ( 'NONE',  ( -35.70801684808192533, -278.6321335968947324, -346.5565930846804008 ) ) ;
#8756=CARTESIAN_POINT ( 'NONE',  ( -79.93762903577183465, -278.9301144844627629, -333.9771067792736972 ) ) ;
#8757=CARTESIAN_POINT ( 'NONE',  ( -108.2891668587348022, -278.6122591604276977, -253.1722562099525931 ) ) ;
#8758=CARTESIAN_POINT ( 'NONE',  ( 18.49961812233036440, -276.8390932206337425, -220.7507943679397044 ) ) ;
#8759=CARTESIAN_POINT ( 'NONE',  ( 30.89892398482169611, -293.0906787496973607, -234.5781795128535236 ) ) ;
#8760=CARTESIAN_POINT ( 'NONE',  ( 34.84375156129817697, -285.8085040057915194, -290.2835716721302788 ) ) ;
#8761=CARTESIAN_POINT ( 'NONE',  ( -56.01269552987617573, -293.4158586769929116, -196.4295796115042947 ) ) ;
#8762=CARTESIAN_POINT ( 'NONE',  ( -31.59176960551908664, -293.8983255112391362, -343.4947136604575348 ) ) ;
#8763=CARTESIAN_POINT ( 'NONE',  ( -18.21904986708069885, -294.4655268256878458, -340.8338909781096504 ) ) ;
#8764=CARTESIAN_POINT ( 'NONE',  ( -53.33831859497281158, -292.9314303861448252, -195.3028325744306528 ) ) ;
#8765=CARTESIAN_POINT ( 'NONE',  ( 25.65107458195391388, -282.7135141998683139, -307.5529823898622794 ) ) ;
#8767=CARTESIAN_POINT ( 'NONE',  ( -105.3947844530108426, -272.0718114215542300, -234.7272850809890485 ) ) ;
#8768=CARTESIAN_POINT ( 'NONE',  ( 25.45706201712810213, -287.6152167461628437, -225.9579244848563064 ) ) ;
#8769=CARTESIAN_POINT ( 'NONE',  ( -48.86163953578493846, -289.5281946450620012, -346.5270388850194081 ) ) ;
#8771=CARTESIAN_POINT ( 'NONE',  ( 9.040652902875526920, -287.0427918944928933, -213.9628483815318418 ) ) ;
#8773=CARTESIAN_POINT ( 'NONE',  ( 151.8583176937316068, 206.6135508955686078, -215.5781253388939263 ) ) ;
#8774=CARTESIAN_POINT ( 'NONE',  ( 196.0033876829498070, 282.0444326092349456, -110.2343316263346225 ) ) ;
#8775=CARTESIAN_POINT ( 'NONE',  ( -1.399799699311389034, -275.7600219461334063, -334.1427038040458228 ) ) ;
#8776=CARTESIAN_POINT ( 'NONE',  ( -103.4155531380339852, -277.0432582185592878, -302.2350717642920586 ) ) ;
#8777=CARTESIAN_POINT ( 'NONE',  ( -94.12679818157711509, -272.9261527909770280, -218.3686165279408442 ) ) ;
#8778=CARTESIAN_POINT ( 'NONE',  ( -75.53332942106331416, -209.1016162018847240, -354.5739361953594653 ) ) ;
#8779=CARTESIAN_POINT ( 'NONE',  ( -101.6913368279449656, -276.6894594216915380, -311.8392469835088150 ) ) ;
#8780=CARTESIAN_POINT ( 'NONE',  ( 32.49423713272408776, -295.7003341314283489, -300.4426475121769613 ) ) ;
#8781=CARTESIAN_POINT ( 'NONE',  ( -7.250624518972343502, -292.9501922423569908, -203.7839776825608169 ) ) ;
#8782=CARTESIAN_POINT ( 'NONE',  ( -62.80120326237123862, -298.5318025517080969, -197.8630316601054631 ) ) ;
#8783=CARTESIAN_POINT ( 'NONE',  ( -72.61013518624845631, -288.2143746204559989, -334.8388735834182626 ) ) ;
#8784=CARTESIAN_POINT ( 'NONE',  ( -26.22707059741377833, -298.6801596957266156, -193.4217551796634496 ) ) ;
#8785=CARTESIAN_POINT ( 'NONE',  ( -90.04733525985048459, -297.4484094351386716, -219.7802008165302254 ) ) ;
#8788=CARTESIAN_POINT ( 'NONE',  ( -98.28127178982454382, -281.0771087560849537, -225.6662065153367678 ) ) ;
#8789=CARTESIAN_POINT ( 'NONE',  ( -91.53455490465863420, -280.3367473239707692, -220.9914859695152813 ) ) ;
#8790=CARTESIAN_POINT ( 'NONE',  ( -94.43441569393428381, -279.6246213802590432, -320.5048697812906653 ) ) ;
#8791=CARTESIAN_POINT ( 'NONE',  ( -38.06997183454770095, -272.5227396771578583, -196.6713807399352731 ) ) ;
#8794=CARTESIAN_POINT ( 'NONE',  ( -69.74220494141258087, -279.7799096825131073, -204.9316220995302160 ) ) ;
#8795=CARTESIAN_POINT ( 'NONE',  ( 39.54591934718346380, -276.3649922940036845, -271.1597390275266548 ) ) ;
#8796=CARTESIAN_POINT ( 'NONE',  ( 34.16371971671559038, -277.8442825702844630, -292.9879954013105134 ) ) ;
#8797=CARTESIAN_POINT ( 'NONE',  ( -104.4666875413394820, -276.6508195428239674, -306.8692315493541400 ) ) ;
#8800=CARTESIAN_POINT ( 'NONE',  ( 37.24687449644227399, -283.6690582316879841, -281.0826541780784851 ) ) ;
#8801=CARTESIAN_POINT ( 'NONE',  ( -34.84154728004926938, -291.2815254128081506, -197.2423723484104698 ) ) ;
#8802=CARTESIAN_POINT ( 'NONE',  ( 37.62212644343407675, -286.6854549103712770, -253.1638780941509594 ) ) ;
#8803=CARTESIAN_POINT ( 'NONE',  ( -69.46902822664068822, -281.7207405807442910, -337.0520136108823408 ) ) ;
#8804=CARTESIAN_POINT ( 'NONE',  ( -71.69994364539020637, -282.0902996228408028, -335.4371198632049982 ) ) ;
#8805=CARTESIAN_POINT ( 'NONE',  ( 17.97679359525062992, -284.9324314844240575, -220.5306518247968199 ) ) ;
#8806=CARTESIAN_POINT ( 'NONE',  ( 25.46818044768311395, -282.2361618086653152, -232.2883337444480674 ) ) ;
#8807=CARTESIAN_POINT ( 'NONE',  ( 5.216658706816619251, -58.13088329177625013, -354.5881770784516220 ) ) ;
#8808=CARTESIAN_POINT ( 'NONE',  ( 19.17630823742029023, -280.6540638180429710, -321.5475374455423321 ) ) ;
#8809=CARTESIAN_POINT ( 'NONE',  ( -9.116443863000283088, -296.6833939340781967, -339.9023675921752670 ) ) ;
#8810=CARTESIAN_POINT ( 'NONE',  ( -94.52759281103743660, -278.5611422399646813, -315.9186369926540578 ) ) ;
#8811=CARTESIAN_POINT ( 'NONE',  ( -99.49526654323518926, -287.1243932118238718, -227.9966482142457664 ) ) ;
#8812=CARTESIAN_POINT ( 'NONE',  ( -17.03751392358046601, -294.2324725654883082, -197.5802536154615154 ) ) ;
#8813=CARTESIAN_POINT ( 'NONE',  ( 37.34335267491378829, -273.6401488032504403, -277.2272329538114946 ) ) ;
#8815=CARTESIAN_POINT ( 'NONE',  ( -78.05952675160035881, -288.7814817325821082, -335.5861958324853163 ) ) ;
#8816=CARTESIAN_POINT ( 'NONE',  ( 19.10145958894884544, -291.2838839168877598, -222.8152439431893299 ) ) ;
#8818=CARTESIAN_POINT ( 'NONE',  ( -110.6493762780347083, -277.3053443508624696, -265.1430633173523006 ) ) ;
#8819=CARTESIAN_POINT ( 'NONE',  ( -88.96802036710012374, -295.4573042168419761, -216.9453142737689291 ) ) ;
#8820=CARTESIAN_POINT ( 'NONE',  ( -68.95503579391693449, -290.7920145428935257, -336.7074855378030520 ) ) ;
#8821=LINE ( 'NONE', #1729, #15468 ) ;
#8823=CARTESIAN_POINT ( 'NONE',  ( 37.10319471813262737, -292.2442045832531221, -287.1731007256407793 ) ) ;
#8824=CARTESIAN_POINT ( 'NONE',  ( 20.96026054497454183, -288.5218459346884856, -225.1137777390445649 ) ) ;
#8825=CARTESIAN_POINT ( 'NONE',  ( -79.01963551630201721, -289.7387365723944868, -206.7614420887572919 ) ) ;
#8826=CARTESIAN_POINT ( 'NONE',  ( 36.13983601538115664, -288.9142125528392171, -265.5300800589415076 ) ) ;
#8829=CARTESIAN_POINT ( 'NONE',  ( 3.713658600522237840, -289.2871051723014375, -330.9784599611290332 ) ) ;
#8830=CARTESIAN_POINT ( 'NONE',  ( -0.2467297892711489415, -296.5413047835233442, -335.9684294254646488 ) ) ;
#8833=CARTESIAN_POINT ( 'NONE',  ( -71.71447333732866980, -290.7013379670577820, -338.8192890217146669 ) ) ;
#8834=CARTESIAN_POINT ( 'NONE',  ( -85.72884325207586187, -277.4067713215529807, -212.5255641192478038 ) ) ;
#8835=CARTESIAN_POINT ( 'NONE',  ( -113.6966930768198978, -279.0128603038735946, -260.1748714753144895 ) ) ;
#8836=CARTESIAN_POINT ( 'NONE',  ( -73.75189508746018419, -279.2490262573203381, -202.5225623299791664 ) ) ;
#8837=CARTESIAN_POINT ( 'NONE',  ( -46.95670227955788789, -283.9300092139282583, -195.9278233555905899 ) ) ;
#8839=CARTESIAN_POINT ( 'NONE',  ( 19.80184082204314677, -279.0307227091901723, -222.9548719994163548 ) ) ;
#8840=CARTESIAN_POINT ( 'NONE',  ( -68.38257587989305364, -281.4597367734060072, -338.6500801736776793 ) ) ;
#8842=CARTESIAN_POINT ( 'NONE',  ( -113.0268343713029111, -277.1597560483435814, -260.2404540504937245 ) ) ;
#8843=CARTESIAN_POINT ( 'NONE',  ( -106.8689884798507563, -274.2955077142498794, -246.2503093870082012 ) ) ;
#8844=CARTESIAN_POINT ( 'NONE',  ( -97.32998023095191797, -284.1147755196226967, -222.5814281366277498 ) ) ;
#8845=CARTESIAN_POINT ( 'NONE',  ( -110.5035570052937004, -273.3907877843992082, -267.6414315660219359 ) ) ;
#8846=CARTESIAN_POINT ( 'NONE',  ( -95.59038497043366078, -274.6493756253075276, -220.8869774345099017 ) ) ;
#8847=CARTESIAN_POINT ( 'NONE',  ( -19.01573596297292568, -276.4763902001100178, -341.0452500356694259 ) ) ;
#8848=CARTESIAN_POINT ( 'NONE',  ( 4.965005543248443232, -296.4805289413608875, -332.2896518079440966 ) ) ;
#8849=CARTESIAN_POINT ( 'NONE',  ( -102.3001188250270843, -290.1757706292937087, -311.8041704862518486 ) ) ;
#8850=CARTESIAN_POINT ( 'NONE',  ( -71.82736713252313621, -277.6798704602044836, -203.1154033255956506 ) ) ;
#8851=CARTESIAN_POINT ( 'NONE',  ( -107.7322323306574674, -289.9856949406647573, -301.7040101081535681 ) ) ;
#8852=CARTESIAN_POINT ( 'NONE',  ( -34.58110174421783967, -288.0755005284748904, -343.5941064689160953 ) ) ;
#8853=CARTESIAN_POINT ( 'NONE',  ( 0.7080000526884929757, -290.5589297708508525, -205.6703330189166365 ) ) ;
#8854=ORIENTED_EDGE ( 'NONE', *, *, #7938, .F. ) ;
#8856=CARTESIAN_POINT ( 'NONE',  ( -108.7694091725905423, -290.2623174363489511, -254.9965215831203693 ) ) ;
#8858=CARTESIAN_POINT ( 'NONE',  ( -26.66572345227279683, -287.1259050288720687, -194.2890767046102098 ) ) ;
#8859=CARTESIAN_POINT ( 'NONE',  ( -6.998514795304313196, -294.9805209788416391, -207.2794874003663779 ) ) ;
#8860=CARTESIAN_POINT ( 'NONE',  ( -33.45876391898881508, -294.0631770539525291, -347.0406373393321360 ) ) ;
#8861=CARTESIAN_POINT ( 'NONE',  ( 36.71866745073334215, -283.1090817045886752, -289.5538308758492576 ) ) ;
#8862=CARTESIAN_POINT ( 'NONE',  ( -44.02226279016083765, -285.7986538926571143, -197.6674450321480094 ) ) ;
#8863=CARTESIAN_POINT ( 'NONE',  ( 35.10900311050138356, -276.7047319330010851, -257.9520013652513626 ) ) ;
#8864=CARTESIAN_POINT ( 'NONE',  ( 36.34153764730793057, -291.4171529309782045, -258.3383596302508636 ) ) ;
#8865=CARTESIAN_POINT ( 'NONE',  ( 20.17619755686089889, -273.7068011220162589, -224.7469019056188131 ) ) ;
#8866=ORIENTED_EDGE ( 'NONE', *, *, #27281, .F. ) ;
#8867=CARTESIAN_POINT ( 'NONE',  ( 121.1498776811041438, 150.0802918209077177, -263.8330885344481658 ) ) ;
#8868=CARTESIAN_POINT ( 'NONE',  ( 34.43024595411311140, -293.5715544377029005, -298.1915338441905305 ) ) ;
#8869=CARTESIAN_POINT ( 'NONE',  ( 28.92919003607481798, -289.0192275503286510, -236.3435088388247607 ) ) ;
#8870=CARTESIAN_POINT ( 'NONE',  ( -104.9874654316503921, -298.1018962433801107, -234.1161284526125996 ) ) ;
#8871=CARTESIAN_POINT ( 'NONE',  ( 15.09684731903779031, -287.4681782359988347, -219.4288942946917302 ) ) ;
#8872=CARTESIAN_POINT ( 'NONE',  ( -105.9598608242558839, -278.0562936677613948, -235.8281145685863578 ) ) ;
#8873=CARTESIAN_POINT ( 'NONE',  ( -34.97187626212824085, -292.7325605633918144, -193.4864427115071805 ) ) ;
#8874=CARTESIAN_POINT ( 'NONE',  ( 26.11635329509505965, -285.1391090912272830, -228.9681121035368676 ) ) ;
#8875=CARTESIAN_POINT ( 'NONE',  ( 21.35428108204349584, -294.5569597582612005, -320.1659980786425308 ) ) ;
#8876=CARTESIAN_POINT ( 'NONE',  ( -77.27026606787596563, -291.8335902719472301, -209.2235917918601729 ) ) ;
#8879=CARTESIAN_POINT ( 'NONE',  ( 189.5630867785912983, 267.9798697569148658, -137.6296589467733611 ) ) ;
#8880=CARTESIAN_POINT ( 'NONE',  ( 38.28551502962600495, -288.9440476537624249, -260.2007990974250333 ) ) ;
#8881=CARTESIAN_POINT ( 'NONE',  ( 25.18497378105905682, -291.6952119285918457, -320.2651865833026363 ) ) ;
#8884=CARTESIAN_POINT ( 'NONE',  ( -89.12232278051294543, -282.7215225026916414, -322.3264413919608842 ) ) ;
#8885=CARTESIAN_POINT ( 'NONE',  ( -114.3565631923106025, -278.2392709018845380, -268.7304571307972765 ) ) ;
#8886=CARTESIAN_POINT ( 'NONE',  ( -3.541737745414301308, -282.4994331406393826, -203.5816871522339113 ) ) ;
#8887=CARTESIAN_POINT ( 'NONE',  ( -10.80946628091583506, -93.01466741719902132, -358.5508527417753726 ) ) ;
#8889=CARTESIAN_POINT ( 'NONE',  ( -64.32202481136863526, -284.2816168551030955, -198.8581214070207182 ) ) ;
#8890=CARTESIAN_POINT ( 'NONE',  ( 35.89309306655286491, -285.7594006460940932, -284.8670212524891667 ) ) ;
#8891=CARTESIAN_POINT ( 'NONE',  ( -29.98280919162694147, -276.0047682608227433, -194.9545386671636891 ) ) ;
#8892=CARTESIAN_POINT ( 'NONE',  ( -92.79520295629198756, -297.7212822135711008, -222.7719506575992057 ) ) ;
#8893=CARTESIAN_POINT ( 'NONE',  ( 31.03828969269414628, -292.5963944860451988, -297.4339066869242743 ) ) ;
#8894=CARTESIAN_POINT ( 'NONE',  ( -114.1095749408321041, -279.2595770265206170, -265.8882907956013923 ) ) ;
#8895=CARTESIAN_POINT ( 'NONE',  ( 35.35400940667743441, -275.6399870532713408, -277.0194822890528599 ) ) ;
#8896=CARTESIAN_POINT ( 'NONE',  ( -109.8142680483750411, -273.9493332498915379, -245.2768717625827151 ) ) ;
#8897=CARTESIAN_POINT ( 'NONE',  ( -98.56499441528772820, -276.8547046792191964, -316.5692621096710013 ) ) ;
#8899=CARTESIAN_POINT ( 'NONE',  ( -21.34504598263349351, -274.8469608215774542, -343.6878356007484854 ) ) ;
#8900=CARTESIAN_POINT ( 'NONE',  ( -110.2563722018130363, -298.2687163366159666, -247.3370227819160334 ) ) ;
#8904=CARTESIAN_POINT ( 'NONE',  ( -59.02650409185191194, -284.4189734439064523, -340.4430138669884514 ) ) ;
#8905=CARTESIAN_POINT ( 'NONE',  ( -63.54131630630689642, -285.1491385968288910, -341.6882104878432642 ) ) ;
#8906=CARTESIAN_POINT ( 'NONE',  ( -79.36110500714751481, -284.8169325023645797, -210.4804006476250606 ) ) ;
#8907=CARTESIAN_POINT ( 'NONE',  ( -107.0262733061681928, -276.6304648514791893, -294.8164459674502496 ) ) ;
#8908=CARTESIAN_POINT ( 'NONE',  ( -109.6226419287274467, -286.1924071183014462, -287.3378962287779359 ) ) ;
#8909=CARTESIAN_POINT ( 'NONE',  ( -91.79622016618665725, -277.7373736914510687, -220.7081925858389013 ) ) ;
#8910=CARTESIAN_POINT ( 'NONE',  ( 30.56955190731863325, -277.0017030970631140, -298.1058157186008657 ) ) ;
#8912=CARTESIAN_POINT ( 'NONE',  ( -85.35532082060400683, -273.8599807757759095, -215.2239030790885010 ) ) ;
#8913=CARTESIAN_POINT ( 'NONE',  ( 20.93693692956661678, -281.6774159029168345, -220.2635816944431610 ) ) ;
#8914=CARTESIAN_POINT ( 'NONE',  ( -27.37385590155814086, -283.4212073084198664, -346.7044687932805118 ) ) ;
#8918=CARTESIAN_POINT ( 'NONE',  ( 31.57840887707521205, -289.0022579166670198, -238.7654938221631937 ) ) ;
#8919=CARTESIAN_POINT ( 'NONE',  ( -102.9174208145260394, -295.3091681613669834, -302.9167584809586629 ) ) ;
#8920=CARTESIAN_POINT ( 'NONE',  ( -34.95525496102173690, -291.4299447735451736, -193.4869571376665078 ) ) ;
#8921=CARTESIAN_POINT ( 'NONE',  ( 34.96067494489496141, -286.2190965345413360, -284.6766792354404743 ) ) ;
#8922=CARTESIAN_POINT ( 'NONE',  ( -8.000108060882192618, -287.2349262631291822, -337.9022211624149463 ) ) ;
#8923=CARTESIAN_POINT ( 'NONE',  ( -77.27791800869859173, -286.7089660836688836, -208.7197317341725125 ) ) ;
#8924=CARTESIAN_POINT ( 'NONE',  ( -96.37098770878827736, -275.9170559299510614, -316.6271299238869119 ) ) ;
#8925=CARTESIAN_POINT ( 'NONE',  ( -51.55625700102394404, -287.6309210686104620, -345.2235704297799543 ) ) ;
#8926=CARTESIAN_POINT ( 'NONE',  ( -31.07697561381440110, -288.1314472800266344, -195.6102673928900231 ) ) ;
#8927=CARTESIAN_POINT ( 'NONE',  ( -12.84584470881603302, -286.7344887958782351, -341.4788733514471915 ) ) ;
#8928=CARTESIAN_POINT ( 'NONE',  ( -38.87803493658780241, -284.0131123915988383, -343.5928279372172938 ) ) ;
#8929=CARTESIAN_POINT ( 'NONE',  ( -66.33245954898512764, -293.6736317099993130, -201.0100956657519760 ) ) ;
#8932=CARTESIAN_POINT ( 'NONE',  ( -79.83577301879198274, -299.4029969769662785, -207.8196567918878941 ) ) ;
#8933=CARTESIAN_POINT ( 'NONE',  ( 2.801108927935374027, -279.8028150310561273, -209.1353286392399866 ) ) ;
#8934=CARTESIAN_POINT ( 'NONE',  ( 37.56211254831914914, -279.6007446379072690, -274.1584186785586894 ) ) ;
#8935=CARTESIAN_POINT ( 'NONE',  ( 13.28174368073900702, -293.5626728369923057, -328.2367227466242525 ) ) ;
#8936=CARTESIAN_POINT ( 'NONE',  ( 96.24762458268381238, -298.1514505501566532, -196.5983225616837728 ) ) ;
#8937=CARTESIAN_POINT ( 'NONE',  ( -26.84210556344882903, -274.9974281247644967, -344.0569300070972076 ) ) ;
#8938=CARTESIAN_POINT ( 'NONE',  ( 1.846868788303968278, -295.8314366739548404, -332.5945397804495656 ) ) ;
#8940=CARTESIAN_POINT ( 'NONE',  ( -35.51950419750271237, -272.6492990649188073, -193.9590454354158737 ) ) ;
#8941=CARTESIAN_POINT ( 'NONE',  ( -113.1085082524981260, -294.8734690861882086, -263.9335632844120596 ) ) ;
#8942=CARTESIAN_POINT ( 'NONE',  ( -15.39997310808768027, -296.1879093892999890, -340.6567011795976327 ) ) ;
#8944=CARTESIAN_POINT ( 'NONE',  ( -86.59114713265333307, -296.5606627246945095, -324.4637398811782987 ) ) ;
#8946=CARTESIAN_POINT ( 'NONE',  ( -51.83176867698495727, -283.8878783882207699, -196.3589601016375923 ) ) ;
#8947=CARTESIAN_POINT ( 'NONE',  ( -108.1749450250722191, -296.7857258490046206, -252.6562906329563134 ) ) ;
#8948=CARTESIAN_POINT ( 'NONE',  ( -113.4874264431697100, -284.6995975975067381, -258.5715010272343193 ) ) ;
#8949=CARTESIAN_POINT ( 'NONE',  ( 28.02831123012526149, -282.9700742869529790, -232.4655270653493915 ) ) ;
#8950=CARTESIAN_POINT ( 'NONE',  ( -104.0200194314797670, -284.7202859603532943, -231.7876577858365863 ) ) ;
#8951=CARTESIAN_POINT ( 'NONE',  ( -106.8245585493610719, -288.1875797782519157, -298.2880949520864533 ) ) ;
#8952=CARTESIAN_POINT ( 'NONE',  ( 35.77081079830085031, -279.2666405000204009, -287.0812184334320705 ) ) ;
#8953=CARTESIAN_POINT ( 'NONE',  ( 16.34609039726634450, -285.5196583220530897, -220.1542502294403505 ) ) ;
#8955=CARTESIAN_POINT ( 'NONE',  ( -112.8314841097673167, -289.3017874062621786, -283.9551682165991338 ) ) ;
#8956=DIRECTION ( 'NONE',  ( 0.000000000000000000, 0.000000000000000000, -1.000000000000000000 ) ) ;
#8957=CARTESIAN_POINT ( 'NONE',  ( -111.1750721578119396, -298.1735020312980851, -268.7353858335342238 ) ) ;
#8958=CARTESIAN_POINT ( 'NONE',  ( -111.2528298213950961, -279.7323183535153248, -289.7967852478623172 ) ) ;
#8959=CARTESIAN_POINT ( 'NONE',  ( -6.494570443607216248, -292.6691636014465416, -339.1132917389062982 ) ) ;
#8960=CARTESIAN_POINT ( 'NONE',  ( 13.35283445964067717, -280.4516989608321182, -217.7344739335650843 ) ) ;
#8961=CARTESIAN_POINT ( 'NONE',  ( -53.28717320853930062, -295.4177453959280228, -345.7465435217305298 ) ) ;
#8962=CARTESIAN_POINT ( 'NONE',  ( -65.32097911435121773, -283.7691591568415674, -200.1583840204513365 ) ) ;
#8963=CARTESIAN_POINT ( 'NONE',  ( -106.6737622213088770, -280.9255136201136338, -241.7592681813426623 ) ) ;
#8965=CARTESIAN_POINT ( 'NONE',  ( -82.51433374258961351, -294.7450277702720882, -328.0698767542548353 ) ) ;
#8966=CARTESIAN_POINT ( 'NONE',  ( -93.69472774365132750, -271.2420196176707350, -220.6181314724049685 ) ) ;
#8969=CARTESIAN_POINT ( 'NONE',  ( 31.86880984511438442, -283.8982011302159094, -298.3209482664706229 ) ) ;
#8970=CARTESIAN_POINT ( 'NONE',  ( -97.23741703219596388, -295.4769168562332879, -312.1999939029255415 ) ) ;
#8972=CARTESIAN_POINT ( 'NONE',  ( -37.37352853689063181, -280.5523547857346784, -345.3611179825600175 ) ) ;
#8973=CARTESIAN_POINT ( 'NONE',  ( -49.68320502573006081, -273.0958948290449939, -194.4665000897131790 ) ) ;
#8975=CARTESIAN_POINT ( 'NONE',  ( -93.43847437855436056, -291.0484244716171816, -223.6280952983300949 ) ) ;
#8976=CARTESIAN_POINT ( 'NONE',  ( -98.58045777634879414, -280.6373498300529832, -229.2762995188936941 ) ) ;
#8977=CARTESIAN_POINT ( 'NONE',  ( -8.678730652493355180, -276.0335845328903588, -202.3001930762216318 ) ) ;
#8978=CARTESIAN_POINT ( 'NONE',  ( 37.36529517251588572, -283.3419686120200254, -285.3712902237767821 ) ) ;
#8979=CARTESIAN_POINT ( 'NONE',  ( -30.20860283698491600, -278.9391794219854432, -197.2608520877612364 ) ) ;
#8980=CARTESIAN_POINT ( 'NONE',  ( -81.99013534660765856, -279.6609526058850861, -330.6231946009731359 ) ) ;
#8982=CARTESIAN_POINT ( 'NONE',  ( -31.25794847127400544, -273.9602837596399354, -193.5885507151284344 ) ) ;
#8983=CARTESIAN_POINT ( 'NONE',  ( 7.525080303610641508, -294.5898577112423595, -210.9617391248979175 ) ) ;
#8986=CARTESIAN_POINT ( 'NONE',  ( -33.57666512363037015, -290.2386593933031804, -194.6899213923076388 ) ) ;
#8987=CARTESIAN_POINT ( 'NONE',  ( -57.90667237330372785, -297.4457873953132889, -200.2956528570652495 ) ) ;
#8989=CARTESIAN_POINT ( 'NONE',  ( -35.00124913942655525, -293.6011288634526295, -194.0773181972479335 ) ) ;
#8990=CARTESIAN_POINT ( 'NONE',  ( 31.98288692825981272, -284.4805209788416960, -303.7098442033569654 ) ) ;
#8992=CARTESIAN_POINT ( 'NONE',  ( 14.38895274998998630, -288.7812082887159022, -216.2159241868751849 ) ) ;
#8993=CARTESIAN_POINT ( 'NONE',  ( -5.519584758828873561, -274.6324594877216327, -338.1054399271781676 ) ) ;
#8994=CARTESIAN_POINT ( 'NONE',  ( 19.42202864065373902, -278.1437641275746842, -318.5191214375342952 ) ) ;
#8995=CARTESIAN_POINT ( 'NONE',  ( 28.77655579912167383, -291.1759152057372830, -236.1603807368060473 ) ) ;
#8996=CARTESIAN_POINT ( 'NONE',  ( -22.82641289902340986, -282.0962551499732172, -195.9463751759451213 ) ) ;
#8997=VERTEX_POINT ( 'NONE', #57220 ) ;
#8998=CARTESIAN_POINT ( 'NONE',  ( -3.615388837699111235, -282.2609237244788005, -335.1410392491600874 ) ) ;
#8999=CARTESIAN_POINT ( 'NONE',  ( -113.9030652395410641, -279.6877662628817802, -265.9057974263764095 ) ) ;
#9000=CARTESIAN_POINT ( 'NONE',  ( 22.20486611472177430, -280.9968393556202955, -318.5711761363790515 ) ) ;
#9001=CARTESIAN_POINT ( 'NONE',  ( -35.70447383852102519, -277.9733637830140083, -347.1214468863662432 ) ) ;
#9002=CARTESIAN_POINT ( 'NONE',  ( 22.11308348202614482, -277.7193073687471383, -318.2131265242443305 ) ) ;
#9003=CARTESIAN_POINT ( 'NONE',  ( -67.74223827176244583, -288.1233781216987495, -207.3071070584150277 ) ) ;
#9005=CARTESIAN_POINT ( 'NONE',  ( -111.7230492094858505, -298.6807984470408996, -260.3544738186429868 ) ) ;
#9006=CARTESIAN_POINT ( 'NONE',  ( -109.4806578211212695, -291.4604550107221144, -283.4070697366714739 ) ) ;
#9007=CARTESIAN_POINT ( 'NONE',  ( -99.02185173252895822, -276.0002894747262303, -312.4016424949765565 ) ) ;
#9008=CARTESIAN_POINT ( 'NONE',  ( -82.23567256706812145, -291.4155524855503359, -331.6677672964936505 ) ) ;
#9009=CARTESIAN_POINT ( 'NONE',  ( -90.82811693935741459, -290.6164386047281596, -220.5119404252024538 ) ) ;
#9010=CARTESIAN_POINT ( 'NONE',  ( 25.79761164024652587, -287.6423138074338794, -314.4179579310767281 ) ) ;
#9012=CARTESIAN_POINT ( 'NONE',  ( -108.1653458178780483, -282.6799777510105969, -291.1536097612043932 ) ) ;
#9013=CARTESIAN_POINT ( 'NONE',  ( -108.1873992785075842, -292.7020722548153344, -248.1427604890856742 ) ) ;
#9014=CARTESIAN_POINT ( 'NONE',  ( -111.0127717019655620, -282.9890455435875651, -273.6499541224108043 ) ) ;
#9015=CARTESIAN_POINT ( 'NONE',  ( 35.92208456830006469, -282.9514093775057404, -276.7776406674568648 ) ) ;
#9016=CARTESIAN_POINT ( 'NONE',  ( -113.1258495113986697, -291.3399737695850718, -282.5915274344486647 ) ) ;
#9017=CARTESIAN_POINT ( 'NONE',  ( -72.16455490927796745, -280.0706252229320512, -206.1321741436102855 ) ) ;
#9018=CARTESIAN_POINT ( 'NONE',  ( -66.84824534930707784, -290.4689132258185396, -199.6690214780654173 ) ) ;
#9019=CARTESIAN_POINT ( 'NONE',  ( -18.23209208044610108, -287.0950523456058932, -195.8817975221083145 ) ) ;
#9020=CARTESIAN_POINT ( 'NONE',  ( 16.64724545834705438, -288.8016692722566177, -325.2505412504290803 ) ) ;
#9021=CARTESIAN_POINT ( 'NONE',  ( -54.75839660499872252, -285.9888039149282122, -199.4169394873675571 ) ) ;
#9024=CARTESIAN_POINT ( 'NONE',  ( 5.773560466611446174, -294.4901583558522020, -208.0603974234272755 ) ) ;
#9025=CARTESIAN_POINT ( 'NONE',  ( -53.20346460585856363, -293.9361297981620851, -345.2598379404914226 ) ) ;
#9026=CARTESIAN_POINT ( 'NONE',  ( 7.715752982756542977, -275.4786830379741787, -328.1598987853102471 ) ) ;
#9027=CARTESIAN_POINT ( 'NONE',  ( -57.35518212490794099, -297.1491651875278990, -196.0578615553173734 ) ) ;
#9029=CARTESIAN_POINT ( 'NONE',  ( 19.01924043422573263, -291.3638773980719634, -222.8832059282251237 ) ) ;
#9030=CARTESIAN_POINT ( 'NONE',  ( -108.9556781276153430, -294.5480056551334087, -289.1038563849991192 ) ) ;
#9031=CARTESIAN_POINT ( 'NONE',  ( -107.3851193177741266, -292.0468377927651886, -248.3858999071535436 ) ) ;
#9032=CARTESIAN_POINT ( 'NONE',  ( 33.41866307921315382, -294.8844540275463828, -289.5712681157908150 ) ) ;
#9034=CARTESIAN_POINT ( 'NONE',  ( -76.15785261883388557, -293.5689970977561529, -334.7904234825163599 ) ) ;
#9035=CARTESIAN_POINT ( 'NONE',  ( -96.95722480694192313, -299.1754566296349935, -224.8321829763796700 ) ) ;
#9036=CARTESIAN_POINT ( 'NONE',  ( -75.98274653586904037, -290.5234782358363645, -332.5726762372370899 ) ) ;
#9037=CARTESIAN_POINT ( 'NONE',  ( 20.48499476488876425, -278.1963951982112349, -318.6775765033436301 ) ) ;
#9038=CARTESIAN_POINT ( 'NONE',  ( -97.29991040655650636, -277.8770260836623720, -222.8394250903219529 ) ) ;
#9039=CARTESIAN_POINT ( 'NONE',  ( -35.51787812975899072, -273.4230329873620349, -193.4715689568409402 ) ) ;
#9040=CARTESIAN_POINT ( 'NONE',  ( 22.50089894521741485, -279.0230394027645957, -226.0657631041955256 ) ) ;
#9041=CARTESIAN_POINT ( 'NONE',  ( -106.6825880866542207, -277.3615779648814623, -238.6385575724773105 ) ) ;
#9042=CARTESIAN_POINT ( 'NONE',  ( -109.5269028076874491, -295.4187228101516212, -256.4905491578002739 ) ) ;
#9044=CARTESIAN_POINT ( 'NONE',  ( 2.979259126803790458, -275.2603832868280165, -209.3242943793279665 ) ) ;
#9046=CARTESIAN_POINT ( 'NONE',  ( -102.3915876516510366, -288.0652167971555286, -308.5027731949417102 ) ) ;
#9047=CARTESIAN_POINT ( 'NONE',  ( -62.76365278926252245, -289.3739762372574660, -343.0998545186443494 ) ) ;
#9048=CARTESIAN_POINT ( 'NONE',  ( -64.26771943868617143, -275.7018206849599551, -200.1687961219183478 ) ) ;
#9049=CARTESIAN_POINT ( 'NONE',  ( -111.8704363618436304, -270.6597741443814584, -261.9665886293834092 ) ) ;
#9050=CARTESIAN_POINT ( 'NONE',  ( -94.28637210267525859, -283.0468769499836412, -321.9700062112144678 ) ) ;
#9051=DIRECTION ( 'NONE',  ( 0.000000000000000000, 0.000000000000000000, -1.000000000000000000 ) ) ;
#9052=CARTESIAN_POINT ( 'NONE',  ( -53.04522905397051602, -281.2531631837518944, -343.7511565776249540 ) ) ;
#9054=CARTESIAN_POINT ( 'NONE',  ( -86.18187002024816934, -290.1519657750760643, -215.5043268487193018 ) ) ;
#9055=CARTESIAN_POINT ( 'NONE',  ( -65.54084169259586190, -283.8191963130745421, -201.6356442246963923 ) ) ;
#9056=CYLINDRICAL_SURFACE ( 'NONE', #63911, 1.897123461337413275 ) ;
#9058=CARTESIAN_POINT ( 'NONE',  ( -3.919549599986841937, -290.4927471186967978, -203.2054626566140030 ) ) ;
#9059=CARTESIAN_POINT ( 'NONE',  ( -109.8252022439424849, -279.9703319762656406, -284.3051988763929216 ) ) ;
#9060=CARTESIAN_POINT ( 'NONE',  ( -52.82228976583626689, -284.4512265979993231, -345.4377237466878228 ) ) ;
#9061=CARTESIAN_POINT ( 'NONE',  ( -75.68058511348679929, -271.6249904509796806, -205.1896579433549448 ) ) ;
#9062=CARTESIAN_POINT ( 'NONE',  ( -68.77493573860628828, -285.6270494822316550, -204.4614294105641363 ) ) ;
#9063=CARTESIAN_POINT ( 'NONE',  ( 16.97825691406048065, -277.6840354190537710, -320.0258360862624727 ) ) ;
#9064=CARTESIAN_POINT ( 'NONE',  ( 11.86384937008692120, -277.1506600438700048, -324.5724204139773974 ) ) ;
#9065=CARTESIAN_POINT ( 'NONE',  ( -84.81619400750905413, -285.7069368887969745, -328.4229219205618620 ) ) ;
#9066=ORIENTED_EDGE ( 'NONE', *, *, #72401, .T. ) ;
#9068=CARTESIAN_POINT ( 'NONE',  ( -47.63367391941932283, -295.0128835428789102, -346.6701952930047810 ) ) ;
#9069=CARTESIAN_POINT ( 'NONE',  ( 34.60811349049909325, -289.2751835694746205, -250.4847218052497340 ) ) ;
#9071=CARTESIAN_POINT ( 'NONE',  ( 13.79469577742117181, -291.9094976428775681, -334.5364918783848793 ) ) ;
#9072=CARTESIAN_POINT ( 'NONE',  ( -113.7722961570585625, -277.3854857085858043, -277.2894164562379729 ) ) ;
#9073=CARTESIAN_POINT ( 'NONE',  ( -61.41630709679873945, -290.1445867640960046, -198.0085671765353084 ) ) ;
#9074=CARTESIAN_POINT ( 'NONE',  ( -105.2438747793397624, -286.4545477554837021, -241.5941884883910689 ) ) ;
#9075=CARTESIAN_POINT ( 'NONE',  ( -65.21828083107389773, -281.4429071139934990, -201.7982252296305603 ) ) ;
#9076=CARTESIAN_POINT ( 'NONE',  ( 29.60648202368650317, -288.4954783408682033, -233.4200445227367879 ) ) ;
#9077=CARTESIAN_POINT ( 'NONE',  ( 35.38898843834155628, -283.3165065688847903, -251.9992449447169918 ) ) ;
#9078=CARTESIAN_POINT ( 'NONE',  ( -38.54283052506055185, -277.2335025225759750, -347.3517491677973794 ) ) ;
#9079=CARTESIAN_POINT ( 'NONE',  ( -87.18016726726369825, -295.3736879954219035, -214.7915760252834048 ) ) ;
#9080=CARTESIAN_POINT ( 'NONE',  ( -53.75840807855522030, -279.6805314468577990, -195.0769560434037260 ) ) ;
#9081=CARTESIAN_POINT ( 'NONE',  ( -75.97856087260620939, -299.4523638578721147, -206.6734643332680719 ) ) ;
#9084=CARTESIAN_POINT ( 'NONE',  ( -95.95921662488163406, -280.4090924074130839, -317.1477375740089997 ) ) ;
#9086=CARTESIAN_POINT ( 'NONE',  ( -34.12338131277177666, -272.3319715076768261, -194.4426324905445256 ) ) ;
#9088=CARTESIAN_POINT ( 'NONE',  ( -110.2302281622285847, -277.9844574312039640, -276.0774600598558663 ) ) ;
#9089=CARTESIAN_POINT ( 'NONE',  ( -10.50119546144568083, -275.5996092216494162, -198.5579425985381192 ) ) ;
#9091=CARTESIAN_POINT ( 'NONE',  ( 29.08898020384873462, -280.1091290761240771, -231.8931452900570207 ) ) ;
#9092=CARTESIAN_POINT ( 'NONE',  ( 6.462152538122775347, -290.2083388516452374, -330.0840053592891650 ) ) ;
#9093=CARTESIAN_POINT ( 'NONE',  ( -46.06995541350183743, -299.4634762869117139, -194.5552784217425994 ) ) ;
#9094=CARTESIAN_POINT ( 'NONE',  ( -36.91511479489226133, -299.2624507052767626, -193.7581024177941345 ) ) ;
#9095=CARTESIAN_POINT ( 'NONE',  ( -64.76662492848308261, -293.6933763771612576, -200.7203664096375917 ) ) ;
#9096=CARTESIAN_POINT ( 'NONE',  ( -0.3677987265727220012, -280.5591494301300486, -335.4223125805726227 ) ) ;
#9097=CARTESIAN_POINT ( 'NONE',  ( 35.98134780013140954, -283.3061134356186699, -257.5141400509570531 ) ) ;
#9098=CARTESIAN_POINT ( 'NONE',  ( -103.4762885368125040, -271.0342565457213482, -235.6361918315443802 ) ) ;
#9099=CARTESIAN_POINT ( 'NONE',  ( -91.35048713360309591, -286.8993379835645783, -216.6071289141591478 ) ) ;
#9100=CARTESIAN_POINT ( 'NONE',  ( -90.82766209874905883, -288.7534240805092054, -320.5698635611984173 ) ) ;
#9101=CARTESIAN_POINT ( 'NONE',  ( -106.5399784064848205, -263.2081406146079985, -317.6450301294818246 ) ) ;
#9103=CARTESIAN_POINT ( 'NONE',  ( -17.89195695092106675, -287.3808470759522038, -344.2550540104290917 ) ) ;
#9104=CARTESIAN_POINT ( 'NONE',  ( -37.27225823610147870, -288.7179772498128045, -343.3822290717908459 ) ) ;
#9106=CARTESIAN_POINT ( 'NONE',  ( -114.0452827560740303, -285.6005324968264745, -272.8529630916000315 ) ) ;
#9107=CARTESIAN_POINT ( 'NONE',  ( 24.00445485794711686, -276.4346995311299224, -310.0616403739940097 ) ) ;
#9109=CARTESIAN_POINT ( 'NONE',  ( 37.12510951001195281, -292.2421902434831509, -252.0257212505495090 ) ) ;
#9110=CARTESIAN_POINT ( 'NONE',  ( 37.09522644561252491, -282.4454282303729542, -289.6602565434245093 ) ) ;
#9111=CARTESIAN_POINT ( 'NONE',  ( 28.67695266115447694, -282.5701066125907346, -232.0956605147805476 ) ) ;
#9112=CARTESIAN_POINT ( 'NONE',  ( 21.59656273432573315, -282.5523519239649772, -319.8790486983861570 ) ) ;
#9113=CARTESIAN_POINT ( 'NONE',  ( 13.33510197507002459, -280.7849264556178923, -217.7467716656487937 ) ) ;
#9114=CARTESIAN_POINT ( 'NONE',  ( -67.74223827176246004, -292.9809262143061233, -333.4151289067050357 ) ) ;
#9115=CARTESIAN_POINT ( 'NONE',  ( 25.64300257841772535, -23.00939279306157559, -345.2368619827582279 ) ) ;
#9117=CARTESIAN_POINT ( 'NONE',  ( 36.92881274143096704, -277.6755328978853754, -279.9362686722686817 ) ) ;
#9118=CARTESIAN_POINT ( 'NONE',  ( -96.09881083034818516, -239.5351746575481116, -341.4074303404881903 ) ) ;
#9119=CARTESIAN_POINT ( 'NONE',  ( 9.018223279003795056, -297.9961767976545275, -197.2644819129092468 ) ) ;
#9120=CARTESIAN_POINT ( 'NONE',  ( 26.45720724600711904, -293.6268434591170262, -313.3637495427612976 ) ) ;
#9121=CARTESIAN_POINT ( 'NONE',  ( 85.38584713910209700, 81.22694468296866432, -299.0555890527453471 ) ) ;
#9122=CARTESIAN_POINT ( 'NONE',  ( -23.47448262698475219, -296.7972917440171159, -193.9536260485545256 ) ) ;
#9123=CARTESIAN_POINT ( 'NONE',  ( -45.47058429120745160, -287.5567332815635950, -343.7120665572656435 ) ) ;
#9124=CARTESIAN_POINT ( 'NONE',  ( -109.4940434518397012, -298.1853584393807637, -287.8761787819575488 ) ) ;
#9125=CARTESIAN_POINT ( 'NONE',  ( -67.76704287674850491, -286.9594315245317375, -203.4616262207693183 ) ) ;
#9127=CARTESIAN_POINT ( 'NONE',  ( -93.50911006021783578, -296.7777182059328993, -322.7067802158568952 ) ) ;
#9128=CARTESIAN_POINT ( 'NONE',  ( -80.65758281933071316, -284.1496973153713839, -329.2604653410962783 ) ) ;
#9129=CARTESIAN_POINT ( 'NONE',  ( -51.71100489476024364, -296.6673148526487580, -195.0639097959698347 ) ) ;
#9130=CARTESIAN_POINT ( 'NONE',  ( -11.21778715862602915, -293.1867848522107920, -198.0438698485044995 ) ) ;
#9131=CARTESIAN_POINT ( 'NONE',  ( 17.44137971370090057, -293.3012842422797348, -216.2644325114591766 ) ) ;
#9132=CARTESIAN_POINT ( 'NONE',  ( -83.83066911307926716, -291.5594250562043044, -214.0781208413714580 ) ) ;
#9135=CARTESIAN_POINT ( 'NONE',  ( -104.1753700635891846, -298.8825151260207917, -234.5627023305806631 ) ) ;
#9136=CARTESIAN_POINT ( 'NONE',  ( 27.30544482081423041, -274.8895997679970264, -311.5541567216604903 ) ) ;
#9139=CARTESIAN_POINT ( 'NONE',  ( -84.83332288771921981, -277.1944949473821680, -330.9604025014336912 ) ) ;
#9140=CARTESIAN_POINT ( 'NONE',  ( -34.42629273200908102, -296.5691725639474612, -196.6685504366246562 ) ) ;
#9141=CARTESIAN_POINT ( 'NONE',  ( -75.15503193404150295, -281.4033739698395493, -206.4191824871593610 ) ) ;
#9142=CARTESIAN_POINT ( 'NONE',  ( -37.84145811329845088, -275.1980249520919983, -344.6073027684507792 ) ) ;
#9143=CARTESIAN_POINT ( 'NONE',  ( -47.34195471741013250, -299.1274695561657495, -197.5970055555608553 ) ) ;
#9144=CARTESIAN_POINT ( 'NONE',  ( -110.4244668606738031, -273.5651163645595716, -264.9078314618561194 ) ) ;
#9145=CARTESIAN_POINT ( 'NONE',  ( -113.3283667958448717, -274.3120101190713740, -270.3834786793233889 ) ) ;
#9146=CARTESIAN_POINT ( 'NONE',  ( -54.92483659935874130, -271.8472745662669467, -197.0860191318285786 ) ) ;
#9147=CARTESIAN_POINT ( 'NONE',  ( -35.63993590234115061, -295.6816902625537864, -343.4557541938581835 ) ) ;
#9148=CARTESIAN_POINT ( 'NONE',  ( -62.98921826990011397, -290.2862291908141970, -201.3859069991136437 ) ) ;
#9150=CARTESIAN_POINT ( 'NONE',  ( -56.90232548531886891, -277.7900761719059233, -344.8265334085669451 ) ) ;
#9151=CARTESIAN_POINT ( 'NONE',  ( 31.11758006296859946, -275.3808760783071534, -245.0169478399705838 ) ) ;
#9152=CARTESIAN_POINT ( 'NONE',  ( -63.02004936067496033, -284.4094411572768877, -198.2922574883576488 ) ) ;
#9153=CARTESIAN_POINT ( 'NONE',  ( -112.5049693374609490, -298.5614778661650348, -269.6460059547466699 ) ) ;
#9155=CARTESIAN_POINT ( 'NONE',  ( -5.719616189304495002, -285.6760467203123426, -204.3727202851144966 ) ) ;
#9156=CARTESIAN_POINT ( 'NONE',  ( -112.5073296679233579, -282.5570572200399511, -269.9654422040516693 ) ) ;
#9157=CARTESIAN_POINT ( 'NONE',  ( -98.49860391413844241, -276.2200049760867842, -312.0481319462705301 ) ) ;
#9158=CARTESIAN_POINT ( 'NONE',  ( -94.92537007064133547, -276.4847930727288485, -316.2015080090582728 ) ) ;
#9160=CARTESIAN_POINT ( 'NONE',  ( -87.95950376613905064, -281.3449301281473254, -214.9489759980830286 ) ) ;
#9161=CARTESIAN_POINT ( 'NONE',  ( 9.728031657626821982, -275.9216909358538032, -213.9778722357959850 ) ) ;
#9163=CARTESIAN_POINT ( 'NONE',  ( -108.4129980346834827, -271.3054697768196775, -242.7330557397093287 ) ) ;
#9165=CARTESIAN_POINT ( 'NONE',  ( -47.88737891490783483, -281.9186281276775503, -195.8853239550579133 ) ) ;
#9167=CARTESIAN_POINT ( 'NONE',  ( -82.43644798484535841, -287.3623993679281625, -209.6676621444179887 ) ) ;
#9169=CARTESIAN_POINT ( 'NONE',  ( -56.38500114910112160, -289.8067327222232734, -197.7660584288144321 ) ) ;
#9171=CARTESIAN_POINT ( 'NONE',  ( -35.11733266678204757, -296.8755288573426583, -196.9645103397436969 ) ) ;
#9172=CARTESIAN_POINT ( 'NONE',  ( -90.68775549754472820, -289.4253738842709254, -218.7368615088576007 ) ) ;
#9173=CARTESIAN_POINT ( 'NONE',  ( 65.71450562203199297, 45.78484130816451625, -315.1169351998001389 ) ) ;
#9175=CARTESIAN_POINT ( 'NONE',  ( 37.04810059467506989, -285.8168868228125916, -253.3070234639806415 ) ) ;
#9176=CARTESIAN_POINT ( 'NONE',  ( -23.90001074543902249, -284.4777052374152504, -342.9266841951295532 ) ) ;
#9177=CARTESIAN_POINT ( 'NONE',  ( -77.96159486801235516, -283.7541092000960248, -206.1427548461797983 ) ) ;
#9178=CARTESIAN_POINT ( 'NONE',  ( -108.1084758968160457, -290.7892470358717674, -252.3920358492311493 ) ) ;
#9179=CARTESIAN_POINT ( 'NONE',  ( 0.6890442174752087201, -281.9948814677866267, -207.3018416625570239 ) ) ;
#9180=CARTESIAN_POINT ( 'NONE',  ( 21.14513809291120694, -282.9710290070006522, -314.3351112133436231 ) ) ;
#9181=CARTESIAN_POINT ( 'NONE',  ( -12.73644950063787817, -290.7139001104780505, -341.6407181709393512 ) ) ;
#9182=CARTESIAN_POINT ( 'NONE',  ( -36.54275480140048415, -298.2285753783489781, -193.3610960453318341 ) ) ;
#9185=CARTESIAN_POINT ( 'NONE',  ( -26.37811156009245650, -286.9935048667940691, -345.1214946649760691 ) ) ;
#9186=CARTESIAN_POINT ( 'NONE',  ( 34.18425571773870786, -275.9155106654981751, -299.0186854183480136 ) ) ;
#9187=CARTESIAN_POINT ( 'NONE',  ( -19.70750661701979212, -294.2597570172372912, -197.7757371491893821 ) ) ;
#9189=CARTESIAN_POINT ( 'NONE',  ( -106.6379572354042296, -280.6233781216988064, -303.7686719486574702 ) ) ;
#9190=CARTESIAN_POINT ( 'NONE',  ( -96.50212868765615326, -275.9170559266127043, -316.7299881841029219 ) ) ;
#9192=CARTESIAN_POINT ( 'NONE',  ( -86.92607734711852174, -295.7757042214179819, -212.4311402268074005 ) ) ;
#9193=CARTESIAN_POINT ( 'NONE',  ( -90.26468574689654645, -272.6271513255361469, -219.9141414218865123 ) ) ;
#9194=CARTESIAN_POINT ( 'NONE',  ( -109.9633529955325457, -292.2397244722101846, -257.5472157442295043 ) ) ;
#9195=CARTESIAN_POINT ( 'NONE',  ( -96.95986742359423260, -292.0867545243746690, -227.7420105527843930 ) ) ;
#9196=CARTESIAN_POINT ( 'NONE',  ( -108.7327328792310084, -286.0572837542106868, -289.9356755233485501 ) ) ;
#9197=CARTESIAN_POINT ( 'NONE',  ( 17.05726805101543420, -294.2340589614796045, -216.6269770537394379 ) ) ;
#9198=CARTESIAN_POINT ( 'NONE',  ( 37.57556621645260009, -294.6712314311852765, -254.7824184169341777 ) ) ;
#9199=CARTESIAN_POINT ( 'NONE',  ( 29.48920500658742228, -293.7806032168152228, -299.7316835774735182 ) ) ;
#9200=CARTESIAN_POINT ( 'NONE',  ( 25.18780854749623188, -288.9919255907174147, -228.8538412119010275 ) ) ;
#9201=CARTESIAN_POINT ( 'NONE',  ( 17.82775891794059220, -282.4559784356180785, -324.1525821193869206 ) ) ;
#9202=CARTESIAN_POINT ( 'NONE',  ( -79.79536173366994944, -295.5633072455308934, -207.7922159327702332 ) ) ;
#9203=CARTESIAN_POINT ( 'NONE',  ( -57.75389097702219487, -285.6290778144822866, -196.0606156211788402 ) ) ;
#9204=CARTESIAN_POINT ( 'NONE',  ( 23.60964851202093584, -276.9435381818844348, -227.2486325963364493 ) ) ;
#9206=CARTESIAN_POINT ( 'NONE',  ( -107.7314009193064095, -283.6228332469245856, -249.3902518422579533 ) ) ;
#9207=CARTESIAN_POINT ( 'NONE',  ( 22.52985302956614433, -286.1695701984517655, -315.5318803675999106 ) ) ;
#9208=CARTESIAN_POINT ( 'NONE',  ( -112.9763733789620659, -276.7481522989206155, -265.9224604803757757 ) ) ;
#9210=CARTESIAN_POINT ( 'NONE',  ( -103.5385673699460085, -284.4783959399725859, -239.3225538553712397 ) ) ;
#9211=CARTESIAN_POINT ( 'NONE',  ( -112.3320105730065990, -279.9545684241080608, -254.6625159821743694 ) ) ;
#9212=CARTESIAN_POINT ( 'NONE',  ( 33.64642815502740092, -286.2369473492973384, -241.0073738777431060 ) ) ;
#9213=CARTESIAN_POINT ( 'NONE',  ( -8.819951329815337360, -296.4339930625933448, -338.6719415027869218 ) ) ;
#9214=CARTESIAN_POINT ( 'NONE',  ( -20.28514319310341563, -278.4368442357993558, -344.6817803636983513 ) ) ;
#9215=CARTESIAN_POINT ( 'NONE',  ( 19.52196237491152075, -277.5667152321353797, -321.5649270622869835 ) ) ;
#9216=CARTESIAN_POINT ( 'NONE',  ( -70.45469727677706828, -277.3347523296615122, -335.4190108500763472 ) ) ;
#9217=CARTESIAN_POINT ( 'NONE',  ( -93.23065889118245764, -299.2464325808889498, -220.5971479192537004 ) ) ;
#9218=CARTESIAN_POINT ( 'NONE',  ( -16.64088514526811124, -284.3199027410548752, -198.3937629426661431 ) ) ;
#9219=CARTESIAN_POINT ( 'NONE',  ( -59.77214241290157304, -290.9381350083733082, -343.1849854490653797 ) ) ;
#9220=CARTESIAN_POINT ( 'NONE',  ( -20.79170200569873472, -293.7551444382265231, -341.8299909895254132 ) ) ;
#9222=CARTESIAN_POINT ( 'NONE',  ( 34.85822803511160828, -293.3672232948167107, -281.6104102700148246 ) ) ;
#9223=CARTESIAN_POINT ( 'NONE',  ( -84.08885930499720018, -292.5065349058130550, -209.4978330762367591 ) ) ;
#9224=CARTESIAN_POINT ( 'NONE',  ( -37.01618781890024223, -280.7077496143334656, -197.2599093036648128 ) ) ;
#9226=CARTESIAN_POINT ( 'NONE',  ( 19.11967835457857845, -297.6638056878800853, -193.6802856397917481 ) ) ;
#9227=CARTESIAN_POINT ( 'NONE',  ( 39.60060493744474286, -288.2183452828665509, -271.5414338850840181 ) ) ;
#9228=CARTESIAN_POINT ( 'NONE',  ( 19.61146230834608417, -288.5896331962988484, -322.1695704097429598 ) ) ;
#9229=CARTESIAN_POINT ( 'NONE',  ( -35.93731551994839890, -286.4035304601642906, -197.3534800894326509 ) ) ;
#9230=FACE_OUTER_BOUND ( 'NONE', #55636, .T. ) ;
#9231=CARTESIAN_POINT ( 'NONE',  ( -104.8366539456450539, -254.2583971032736940, -325.3939605836368969 ) ) ;
#9232=CARTESIAN_POINT ( 'NONE',  ( -102.1682833893122790, -254.0870747469653566, -324.0649701474447966 ) ) ;
#9234=CARTESIAN_POINT ( 'NONE',  ( -36.47449613086610753, -276.2382106544087037, -343.5299502666913440 ) ) ;
#9235=CARTESIAN_POINT ( 'NONE',  ( -99.44423846440159309, -276.9356955854393050, -309.4110797231923016 ) ) ;
#9236=CARTESIAN_POINT ( 'NONE',  ( -14.82618927689352972, -297.8346270237912563, -193.4244760388092175 ) ) ;
#9237=CARTESIAN_POINT ( 'NONE',  ( 46.66400796352151303, 10.61984656453235587, -329.2320478923130054 ) ) ;
#9238=CARTESIAN_POINT ( 'NONE',  ( -96.68258349367351911, -276.5846228379504055, -318.6719875330187506 ) ) ;
#9239=CARTESIAN_POINT ( 'NONE',  ( -81.26741293479715011, -297.3999401733335617, -332.4294497083434976 ) ) ;
#9241=CARTESIAN_POINT ( 'NONE',  ( -110.0347439241129734, -291.1410984331432132, -263.0324192407556438 ) ) ;
#9242=CARTESIAN_POINT ( 'NONE',  ( -107.6294690725139276, -297.7533807336070026, -239.1845865574373988 ) ) ;
#9243=CARTESIAN_POINT ( 'NONE',  ( -95.95538381259881078, -273.8756416572669536, -220.5638496629271685 ) ) ;
#9244=CARTESIAN_POINT ( 'NONE',  ( -104.9611038077306375, -296.3503672220018075, -297.8677762764351655 ) ) ;
#9247=CARTESIAN_POINT ( 'NONE',  ( -17.70806079349900841, -278.7209958060949475, -343.3257285949125048 ) ) ;
#9248=CARTESIAN_POINT ( 'NONE',  ( -2.925997099835125681, -282.1172802842498299, -339.1877222854670890 ) ) ;
#9249=CARTESIAN_POINT ( 'NONE',  ( -97.89644304253572216, -279.0593592761925379, -311.6812000781450251 ) ) ;
#9250=CARTESIAN_POINT ( 'NONE',  ( -97.98103580883828556, -279.6940580695944050, -316.1737855163179347 ) ) ;
#9251=CARTESIAN_POINT ( 'NONE',  ( -40.78817235996842783, -272.4880299243721424, -196.6982445760002065 ) ) ;
#9254=CARTESIAN_POINT ( 'NONE',  ( -57.11524933343630295, -279.9565163721202339, -200.0901655462288602 ) ) ;
#9255=CARTESIAN_POINT ( 'NONE',  ( 10.43367144330280105, -277.2147819990506150, -330.6094025640717291 ) ) ;
#9256=CARTESIAN_POINT ( 'NONE',  ( 33.32532904734250678, -277.8796050551589474, -295.6374761423203950 ) ) ;
#9257=CARTESIAN_POINT ( 'NONE',  ( -1.758340108244709432, -275.1647528702646923, -337.9808694157658238 ) ) ;
#9260=CARTESIAN_POINT ( 'NONE',  ( 37.77016376036974776, -283.4547181006087726, -264.3101094794230335 ) ) ;
#9261=CARTESIAN_POINT ( 'NONE',  ( -55.04154764649329223, -291.0158151446058810, -199.3729702094652225 ) ) ;
#9262=CARTESIAN_POINT ( 'NONE',  ( 24.62605641101286125, -286.2951263686590551, -224.8275047242626385 ) ) ;
#9263=CARTESIAN_POINT ( 'NONE',  ( -66.98573991443798548, -281.6859368285051346, -338.1923178402363988 ) ) ;
#9264=CARTESIAN_POINT ( 'NONE',  ( -83.17578265238967106, -282.2683916607443280, -327.9991844447695257 ) ) ;
#9265=CARTESIAN_POINT ( 'NONE',  ( 17.04289510117902040, -284.9147758917934539, -219.5128798779178112 ) ) ;
#9266=CARTESIAN_POINT ( 'NONE',  ( 15.53484523709902021, -282.0254844878625704, -219.3846845375686883 ) ) ;
#9267=CARTESIAN_POINT ( 'NONE',  ( 202.9738562182569694, 295.9636489450776367, -54.00000000004089173 ) ) ;
#9268=CARTESIAN_POINT ( 'NONE',  ( 26.04498570800102186, -280.5145684407276576, -312.6525884457160487 ) ) ;
#9269=CARTESIAN_POINT ( 'NONE',  ( 24.09146401314860597, -296.1366013369365078, -313.4064074905962229 ) ) ;
#9270=CARTESIAN_POINT ( 'NONE',  ( -103.8227961372751196, -287.0174945330898595, -235.1740781949551433 ) ) ;
#9272=CARTESIAN_POINT ( 'NONE',  ( -103.3638481591172678, -292.9577530237928613, -233.6134627514234694 ) ) ;
#9273=CARTESIAN_POINT ( 'NONE',  ( 34.79040958219606239, -273.2854874014033726, -249.6336676311344149 ) ) ;
#9274=CARTESIAN_POINT ( 'NONE',  ( -5.702344222117779360, -287.8437307093554978, -340.3833285940913811 ) ) ;
#9275=CARTESIAN_POINT ( 'NONE',  ( 19.97991237435656942, -291.3013309531997947, -223.8580820775575546 ) ) ;
#9277=CARTESIAN_POINT ( 'NONE',  ( -89.44719669208357971, -276.4896035446204792, -322.2625502989038750 ) ) ;
#9278=CARTESIAN_POINT ( 'NONE',  ( -105.8939361676800104, -295.0673922253043315, -241.8750439835143879 ) ) ;
#9279=CARTESIAN_POINT ( 'NONE',  ( -53.50077043607949179, -290.5790032532176497, -342.0558034434805563 ) ) ;
#9282=CARTESIAN_POINT ( 'NONE',  ( 28.96254726950153113, -292.5281954743124970, -308.2362442120626724 ) ) ;
#9283=CARTESIAN_POINT ( 'NONE',  ( 22.62989943797673575, -288.5565931269269981, -227.2651356116299155 ) ) ;
#9284=CARTESIAN_POINT ( 'NONE',  ( -94.87875627210028995, -289.4714041571656367, -220.7079701932398450 ) ) ;
#9286=CARTESIAN_POINT ( 'NONE',  ( 32.39321816517778529, -288.6676917040457511, -246.8575844714772813 ) ) ;
#9288=CARTESIAN_POINT ( 'NONE',  ( 19.64568605195591644, -289.0022081802937919, -316.2418279152250307 ) ) ;
#9289=CARTESIAN_POINT ( 'NONE',  ( 26.72119379197537015, -296.0633791598679636, -310.1373111701892071 ) ) ;
#9291=CARTESIAN_POINT ( 'NONE',  ( 31.33825936494917386, -289.1968139352492244, -304.4082472752643866 ) ) ;
#9292=CARTESIAN_POINT ( 'NONE',  ( -33.96323542717557586, -278.1145699907761468, -195.0816866541901220 ) ) ;
#9293=CARTESIAN_POINT ( 'NONE',  ( -103.5854320905429802, -278.3732943287595276, -309.6767640793804048 ) ) ;
#9295=CARTESIAN_POINT ( 'NONE',  ( -79.89555834670423451, -279.1606471997329777, -206.1495867284706094 ) ) ;
#9296=CARTESIAN_POINT ( 'NONE',  ( -107.3572157436031489, -298.8712320091726156, -244.3338223848977862 ) ) ;
#9297=CARTESIAN_POINT ( 'NONE',  ( -111.5886471288081765, -282.6881124382738335, -259.7596317679280560 ) ) ;
#9299=CARTESIAN_POINT ( 'NONE',  ( -8.750080944692463447, -278.5698607786820276, -201.8528353145363781 ) ) ;
#9300=CARTESIAN_POINT ( 'NONE',  ( -109.1992937345548569, -282.2747094013134870, -291.8880122362516545 ) ) ;
#9302=CARTESIAN_POINT ( 'NONE',  ( -6.869518930715255323, -275.1393295584406928, -340.3334737087832877 ) ) ;
#9304=CARTESIAN_POINT ( 'NONE',  ( -63.80001349355167406, -296.9234865064245810, -339.1950108594052722 ) ) ;
#9305=CARTESIAN_POINT ( 'NONE',  ( -37.32816513526459801, -281.9722845857710922, -347.0650187101471715 ) ) ;
#9306=CARTESIAN_POINT ( 'NONE',  ( -101.6682902808948796, -297.0171056054360292, -305.3682350702949293 ) ) ;
#9307=CARTESIAN_POINT ( 'NONE',  ( 52.84749097760590075, -300.4742676677981308, -193.8345526933532597 ) ) ;
#9308=CARTESIAN_POINT ( 'NONE',  ( 17.30419981504129368, -274.5262934496395815, -221.8515619462640984 ) ) ;
#9309=CARTESIAN_POINT ( 'NONE',  ( 36.44639545423920879, -295.3789794707898295, -256.8615969540347805 ) ) ;
#9310=CARTESIAN_POINT ( 'NONE',  ( 34.04312958210429230, -288.0868973087494851, -299.3684577602278978 ) ) ;
#9311=CARTESIAN_POINT ( 'NONE',  ( -99.05842242463586445, -277.2198575950725967, -226.7679948077680763 ) ) ;
#9312=CARTESIAN_POINT ( 'NONE',  ( -114.0066250333133411, -290.4821002456295673, -262.6348487506654692 ) ) ;
#9313=CARTESIAN_POINT ( 'NONE',  ( -45.40020517645733378, -288.2155034653073358, -343.1517007822778851 ) ) ;
#9314=CARTESIAN_POINT ( 'NONE',  ( 33.58645800185961861, -291.8692495818679049, -294.8962646433143391 ) ) ;
#9317=CARTESIAN_POINT ( 'NONE',  ( -95.82134458623738738, -289.4453256542315103, -314.1783413290849580 ) ) ;
#9319=CARTESIAN_POINT ( 'NONE',  ( -69.70459707143959349, -286.5776924869188065, -200.7374348708920877 ) ) ;
#9320=CARTESIAN_POINT ( 'NONE',  ( -37.37352853689063181, -294.5519495502701375, -200.3611179825600459 ) ) ;
#9321=CARTESIAN_POINT ( 'NONE',  ( 34.22778269782197214, -292.9636815480681662, -298.1213294457143661 ) ) ;
#9322=CARTESIAN_POINT ( 'NONE',  ( 22.15043002687142959, -283.5166811540997855, -318.4856890816274699 ) ) ;
#9323=CARTESIAN_POINT ( 'NONE',  ( -106.9864936730093348, -284.0955080349102104, -292.2381090140426636 ) ) ;
#9324=CARTESIAN_POINT ( 'NONE',  ( -105.6099249115084575, -273.1795651454737595, -234.6305738050200773 ) ) ;
#9325=CARTESIAN_POINT ( 'NONE',  ( 33.98376699622755126, -276.6350916942104163, -252.6432959120383259 ) ) ;
#9326=CARTESIAN_POINT ( 'NONE',  ( 3.153523199933804921, -290.6186907111285223, -207.5943450251776596 ) ) ;
#9327=CARTESIAN_POINT ( 'NONE',  ( -8.802341622391294251, -273.2288335437097544, -202.6856419010590002 ) ) ;
#9330=CARTESIAN_POINT ( 'NONE',  ( 180.5468918863934960, 256.3577768311903355, -167.2605672291198857 ) ) ;
#9331=CARTESIAN_POINT ( 'NONE',  ( -44.18054286001340358, -287.8851514045184103, -196.2359236978707315 ) ) ;
#9332=CARTESIAN_POINT ( 'NONE',  ( -99.74891817102903246, -297.0379659272837785, -315.0244331584569295 ) ) ;
#9333=CARTESIAN_POINT ( 'NONE',  ( -95.85250664052482250, -285.8178224404293815, -226.5389981144259082 ) ) ;
#9334=CARTESIAN_POINT ( 'NONE',  ( -84.73057161874488941, -276.7456623870044155, -330.8200186737783497 ) ) ;
#9335=CARTESIAN_POINT ( 'NONE',  ( 15.36225741254725286, -293.4246494547327302, -214.2915341415307751 ) ) ;
#9336=CARTESIAN_POINT ( 'NONE',  ( 34.76481083387752591, -285.9890037049091802, -293.6195907857422185 ) ) ;
#9337=CARTESIAN_POINT ( 'NONE',  ( 4.219455850647682027, -294.8419587714506633, -335.2190530474730963 ) ) ;
#9338=CARTESIAN_POINT ( 'NONE',  ( -99.73187561860062544, -291.4078247623962739, -232.4196698157836352 ) ) ;
#9341=CARTESIAN_POINT ( 'NONE',  ( 168.1374001854913161, 229.6528827648448328, -190.0556063143384335 ) ) ;
#9342=CARTESIAN_POINT ( 'NONE',  ( -111.8439212269905028, -285.8640842813732093, -286.8573844371703103 ) ) ;
#9343=CARTESIAN_POINT ( 'NONE',  ( -37.30987171927208834, -295.5523547857347353, -195.3611179825600175 ) ) ;
#9345=CARTESIAN_POINT ( 'NONE',  ( -109.2854881134171734, -283.2874891543556828, -284.4436406515244471 ) ) ;
#9346=CARTESIAN_POINT ( 'NONE',  ( -104.9590386008110983, -277.7426348631080941, -307.1529625857808696 ) ) ;
#9347=CARTESIAN_POINT ( 'NONE',  ( 35.73611740963192318, -283.7596727182389031, -286.4751185696181892 ) ) ;
#9348=CARTESIAN_POINT ( 'NONE',  ( 169.7292685188034227, 230.4183104143901062, -191.5860846049169197 ) ) ;
#9349=CARTESIAN_POINT ( 'NONE',  ( -85.74325200706886108, -282.2820553938334456, -329.4872210758128404 ) ) ;
#9350=CARTESIAN_POINT ( 'NONE',  ( 34.25459885592858456, -285.2985038511157541, -249.2016013927953964 ) ) ;
#9351=CARTESIAN_POINT ( 'NONE',  ( 21.77938134748067966, -276.7672742108748025, -222.9590885080746432 ) ) ;
#9352=CARTESIAN_POINT ( 'NONE',  ( -110.1122087153026143, -297.1375724696620750, -263.2999384606431477 ) ) ;
#9354=CARTESIAN_POINT ( 'NONE',  ( 36.11476244439325711, -292.2065457862624953, -268.0391397338300408 ) ) ;
#9355=CARTESIAN_POINT ( 'NONE',  ( -89.13732877151714717, -278.4097586906273705, -327.1988311645158092 ) ) ;
#9356=CARTESIAN_POINT ( 'NONE',  ( -48.60784014164740796, -277.1994615326570965, -342.5379122864406440 ) ) ;
#9357=CARTESIAN_POINT ( 'NONE',  ( -46.11491558741615648, -298.8846996149286497, -194.0993916506022856 ) ) ;
#9358=CARTESIAN_POINT ( 'NONE',  ( -86.90594116065956598, -276.6432078885947590, -328.9530741798733970 ) ) ;
#9359=CARTESIAN_POINT ( 'NONE',  ( 202.9737692553709962, 295.9636489462768054, -68.65455572929471373 ) ) ;
#9360=CARTESIAN_POINT ( 'NONE',  ( -69.88068506323564577, -275.4804950842052449, -337.9488520313279878 ) ) ;
#9362=CARTESIAN_POINT ( 'NONE',  ( 20.93015744612140239, -295.6487743138541191, -319.7878001415969038 ) ) ;
#9366=CARTESIAN_POINT ( 'NONE',  ( -97.77942276236090891, -285.0556220006229751, -311.9406250675800720 ) ) ;
#9367=CARTESIAN_POINT ( 'NONE',  ( -71.26595434794067785, -285.2540185525364222, -338.3546396788050288 ) ) ;
#9368=CARTESIAN_POINT ( 'NONE',  ( 15.10840051377569715, -286.1655619060246067, -219.4407918758481344 ) ) ;
#9369=CARTESIAN_POINT ( 'NONE',  ( -98.64692345768735038, -277.5176028380968205, -229.1837950430018225 ) ) ;
#9370=CARTESIAN_POINT ( 'NONE',  ( -109.8768178802355919, -286.6182510395533996, -254.5054146310430383 ) ) ;
#9371=CARTESIAN_POINT ( 'NONE',  ( -35.62744554201038483, -278.5538885771593414, -196.6752029966957593 ) ) ;
#9372=CARTESIAN_POINT ( 'NONE',  ( -64.43464373333104334, -278.4938122583737368, -338.5340249355006677 ) ) ;
#9374=CARTESIAN_POINT ( 'NONE',  ( -48.89134119960048963, -274.3935443852893741, -198.1670271450167604 ) ) ;
#9376=CARTESIAN_POINT ( 'NONE',  ( 29.14174062027015921, -281.8529327494938457, -231.8369576884314256 ) ) ;
#9378=CARTESIAN_POINT ( 'NONE',  ( 36.53887046323130505, -281.7744392365738690, -248.8386078375712316 ) ) ;
#9379=ORIENTED_EDGE ( 'NONE', *, *, #41133, .F. ) ;
#9381=CARTESIAN_POINT ( 'NONE',  ( 120.8395553409046528, -299.5541904835127980, -197.5480973984245168 ) ) ;
#9382=CARTESIAN_POINT ( 'NONE',  ( 33.91892579954672016, -289.7445942240782415, -296.2476975210049659 ) ) ;
#9383=CARTESIAN_POINT ( 'NONE',  ( -107.6116207925811352, -296.0180866902563821, -249.9959522083234162 ) ) ;
#9384=CARTESIAN_POINT ( 'NONE',  ( 17.42284735118061434, -292.1577082024437004, -216.3031949670192375 ) ) ;
#9385=CARTESIAN_POINT ( 'NONE',  ( 32.50384318475535395, -285.7227723736917255, -246.8598875580085235 ) ) ;
#9386=CARTESIAN_POINT ( 'NONE',  ( 32.87037456973008176, -286.4186139456267597, -292.5678098937314644 ) ) ;
#9387=CARTESIAN_POINT ( 'NONE',  ( 18.06591383834199860, -288.0746774278188695, -222.2245744819838649 ) ) ;
#9388=CARTESIAN_POINT ( 'NONE',  ( -110.5382276462480746, -276.3420841287217513, -286.7094822062604749 ) ) ;
#9389=CARTESIAN_POINT ( 'NONE',  ( 0.3061181238226263757, -286.9596750936422040, -336.6708858315362818 ) ) ;
#9390=CARTESIAN_POINT ( 'NONE',  ( -63.86438439859188065, -287.7064970884492823, -200.1935717889540456 ) ) ;
#9391=CARTESIAN_POINT ( 'NONE',  ( -51.36876014307293303, -287.2309533524947938, -344.2073772716512963 ) ) ;
#9392=CARTESIAN_POINT ( 'NONE',  ( 21.20520556334179929, -283.1094260327879510, -314.3780755328174905 ) ) ;
#9393=CARTESIAN_POINT ( 'NONE',  ( -71.36575023778237892, -293.6041527637054287, -203.3215524616446714 ) ) ;
#9396=CARTESIAN_POINT ( 'NONE',  ( -112.7942526783575516, -298.4097371523959623, -275.2706406738089413 ) ) ;
#9397=CARTESIAN_POINT ( 'NONE',  ( 33.61469190428632459, -280.5139669131145297, -252.4834640556606473 ) ) ;
#9398=CARTESIAN_POINT ( 'NONE',  ( 6.747804008366109940, -280.4522460350520987, -331.0333214281962455 ) ) ;
#9399=CARTESIAN_POINT ( 'NONE',  ( 6.513436402753930210, -293.6702768332052642, -333.5202053665329913 ) ) ;
#9400=CARTESIAN_POINT ( 'NONE',  ( -77.08980148549616729, -271.7512966860838333, -207.9266527333860495 ) ) ;
#9401=CARTESIAN_POINT ( 'NONE',  ( 6.220049248655174168, -274.5359313369930305, -330.7877276881820308 ) ) ;
#9402=CARTESIAN_POINT ( 'NONE',  ( -4.098710172409132824, -295.9195122302720051, -335.9202126317778152 ) ) ;
#9404=CARTESIAN_POINT ( 'NONE',  ( -93.69831990971792379, -271.8343379430217510, -218.7420208060979974 ) ) ;
#9405=CARTESIAN_POINT ( 'NONE',  ( -97.48631844581680639, -294.1639130578289496, -316.8003137591177847 ) ) ;
#9406=CARTESIAN_POINT ( 'NONE',  ( -12.07480611750736799, -293.8126527156005068, -201.1912628995287946 ) ) ;
#9408=CARTESIAN_POINT ( 'NONE',  ( -0.01734373234466295849, -293.3655432072883968, -207.4366064895172599 ) ) ;
#9410=CARTESIAN_POINT ( 'NONE',  ( -112.2710970162148101, -282.4700302973818680, -278.3606356837190106 ) ) ;
#9411=CARTESIAN_POINT ( 'NONE',  ( 14.31627945125103629, -294.3013321230193924, -322.0117731805708559 ) ) ;
#9412=CARTESIAN_POINT ( 'NONE',  ( 38.42557020330212225, -281.7246931477653220, -284.1573547824448269 ) ) ;
#9413=CARTESIAN_POINT ( 'NONE',  ( -17.39608807173466332, -282.2277362880728333, -197.4811704312260758 ) ) ;
#9414=CARTESIAN_POINT ( 'NONE',  ( -107.9050482121129448, -284.6127052516715707, -239.4616675676830653 ) ) ;
#9415=CARTESIAN_POINT ( 'NONE',  ( -107.7662954873343182, -288.2232244660248170, -295.6673384357686700 ) ) ;
#9416=CARTESIAN_POINT ( 'NONE',  ( -20.19161114001082069, -271.7666405000204577, -195.3683826091709363 ) ) ;
#9417=CARTESIAN_POINT ( 'NONE',  ( -24.66797078881636907, -281.3732731368497184, -345.6615672673524955 ) ) ;
#9418=CARTESIAN_POINT ( 'NONE',  ( -14.39624385009643426, -285.0406471295142978, -200.4883300999165954 ) ) ;
#9419=CARTESIAN_POINT ( 'NONE',  ( -112.6188907879411687, -289.6573926183591539, -255.6354476039742849 ) ) ;
#9421=CARTESIAN_POINT ( 'NONE',  ( 16.75931787345694346, -295.8658678766325920, -320.5559410893037011 ) ) ;
#9422=CARTESIAN_POINT ( 'NONE',  ( -103.0894641370723974, -279.4651095680663389, -309.3985989646350276 ) ) ;
#9423=CARTESIAN_POINT ( 'NONE',  ( 5.654382319007485336, -292.4934067197319791, -332.3096068555218494 ) ) ;
#9424=CARTESIAN_POINT ( 'NONE',  ( 11.32306847253002857, -280.4158516843758662, -215.9200692808280451 ) ) ;
#9425=CARTESIAN_POINT ( 'NONE',  ( 34.45225792870877513, -294.0714351290135937, -298.1932503304552142 ) ) ;
#9426=CARTESIAN_POINT ( 'NONE',  ( -43.52360509942221967, -284.0546177066939890, -195.0021606904724081 ) ) ;
#9427=CARTESIAN_POINT ( 'NONE',  ( -35.72831347859996498, -279.0321009685991953, -345.3565492688085783 ) ) ;
#9428=CARTESIAN_POINT ( 'NONE',  ( -15.53415644707979126, -293.8217661629800546, -340.3275428985779740 ) ) ;
#9430=CARTESIAN_POINT ( 'NONE',  ( -112.3496288967640879, -270.6240362761600977, -264.7374179722997951 ) ) ;
#9434=CARTESIAN_POINT ( 'NONE',  ( 3.585205170984413936, -282.5850915640243102, -207.8744732089052718 ) ) ;
#9435=CARTESIAN_POINT ( 'NONE',  ( -58.43198869703611109, -294.8399360726095892, -340.3124451293195420 ) ) ;
#9437=CARTESIAN_POINT ( 'NONE',  ( -20.25526795762938548, -280.3380690714491266, -345.3683826091709648 ) ) ;
#9438=CARTESIAN_POINT ( 'NONE',  ( -94.01923303865451942, -272.4566771834714132, -218.4589795183534022 ) ) ;
#9439=CARTESIAN_POINT ( 'NONE',  ( 38.06792231139792904, -288.7038455710182348, -257.3734082591798824 ) ) ;
#9440=CARTESIAN_POINT ( 'NONE',  ( -109.2763902914211513, -290.5531949438906736, -257.6467586588815379 ) ) ;
#9442=CARTESIAN_POINT ( 'NONE',  ( -43.83125591036727542, -281.4889182350472083, -196.9033676322069084 ) ) ;
#9443=CARTESIAN_POINT ( 'NONE',  ( -68.64019928937229054, -275.2339793804651435, -203.5128137329799074 ) ) ;
#9444=CARTESIAN_POINT ( 'NONE',  ( 5.165534353092529507, -279.4364851505123966, -210.5257979733775358 ) ) ;
#9446=CARTESIAN_POINT ( 'NONE',  ( 9.512021383094186433, -274.5099932745846445, -209.2568727532990067 ) ) ;
#9447=CARTESIAN_POINT ( 'NONE',  ( -69.66456076751934745, -293.5435032731721208, -203.2907444164762580 ) ) ;
#9451=CARTESIAN_POINT ( 'NONE',  ( 35.52287402197072197, -291.4267013884627318, -249.5518240744340801 ) ) ;
#9452=CARTESIAN_POINT ( 'NONE',  ( -110.2497162214860822, -272.1317480020769040, -264.9026157334960772 ) ) ;
#9454=CARTESIAN_POINT ( 'NONE',  ( -113.3184584092758769, -292.1686304840458774, -262.7257586349020357 ) ) ;
#9455=CARTESIAN_POINT ( 'NONE',  ( -37.37352853689063181, -294.5519495502701375, -190.3611179825600175 ) ) ;
#9456=CARTESIAN_POINT ( 'NONE',  ( -33.16108494954359287, -288.1049510632423107, -195.5935759879883449 ) ) ;
#9457=CARTESIAN_POINT ( 'NONE',  ( 36.92228243610966842, -273.6758569549191407, -279.9867987363098791 ) ) ;
#9458=CARTESIAN_POINT ( 'NONE',  ( 21.81121262166312746, -276.8487912599250649, -225.1489165455837735 ) ) ;
#9459=CARTESIAN_POINT ( 'NONE',  ( 30.05242332892795432, -291.2118248548381416, -238.6269397304359359 ) ) ;
#9460=CARTESIAN_POINT ( 'NONE',  ( -33.99394332330222568, -281.9542575672364251, -194.6703126847654346 ) ) ;
#9463=CARTESIAN_POINT ( 'NONE',  ( 1.147934986711255156, -281.8723990899705427, -332.5687598379224710 ) ) ;
#9464=CARTESIAN_POINT ( 'NONE',  ( -113.7698113889289999, -279.5444806902247024, -277.3167785949152631 ) ) ;
#9465=CARTESIAN_POINT ( 'NONE',  ( 23.08020642156183300, -280.9796477978960638, -317.4694837491276758 ) ) ;
#9466=CARTESIAN_POINT ( 'NONE',  ( -93.15465407850270196, -278.7708410684625733, -323.1415971877929678 ) ) ;
#9468=CARTESIAN_POINT ( 'NONE',  ( 3.150145769630703807, -278.0392902086244362, -335.1003557875072829 ) ) ;
#9469=CARTESIAN_POINT ( 'NONE',  ( 27.36219212280431989, -290.4805209788416391, -301.4846348637938149 ) ) ;
#9471=CARTESIAN_POINT ( 'NONE',  ( -108.6151890816451555, -298.8558147292780518, -246.8491257729131121 ) ) ;
#9472=CARTESIAN_POINT ( 'NONE',  ( -110.6145881170797338, -291.5848479143420491, -273.9376898259026802 ) ) ;
#9473=CARTESIAN_POINT ( 'NONE',  ( -5.599580795686239121, -274.6527245038339515, -337.9346838064539043 ) ) ;
#9474=CARTESIAN_POINT ( 'NONE',  ( 0.2379153472877099940, -290.3194023438956037, -336.4641059641636502 ) ) ;
#9475=CARTESIAN_POINT ( 'NONE',  ( -101.2087008305070981, -290.3876129906558390, -234.6917518073010172 ) ) ;
#9476=CARTESIAN_POINT ( 'NONE',  ( 38.49726714829844809, -286.8966162944844882, -257.3229458393884670 ) ) ;
#9478=CARTESIAN_POINT ( 'NONE',  ( -110.6700310492390003, -282.8375507055343405, -279.1334383318287564 ) ) ;
#9479=CARTESIAN_POINT ( 'NONE',  ( -96.74268996601836079, -291.7977083417767972, -314.9063381743656578 ) ) ;
#9480=CARTESIAN_POINT ( 'NONE',  ( -103.6448513711170278, -282.5993002788165995, -302.6435727770219160 ) ) ;
#9481=CARTESIAN_POINT ( 'NONE',  ( 22.50541189448504653, -282.2754232012916304, -227.7047390776429552 ) ) ;
#9482=CARTESIAN_POINT ( 'NONE',  ( 38.74047069050961767, -288.3652710480009205, -260.1472305566273349 ) ) ;
#9483=CARTESIAN_POINT ( 'NONE',  ( -83.48145137529853343, -279.8922531219755001, -213.6466087886844036 ) ) ;
#9484=CARTESIAN_POINT ( 'NONE',  ( -2.224125328174093141, -291.3013735828918698, -202.2673093764281873 ) ) ;
#9485=CARTESIAN_POINT ( 'NONE',  ( -32.32718939472812991, -286.9166714291579297, -193.6732539625215850 ) ) ;
#9486=CARTESIAN_POINT ( 'NONE',  ( 0.6943330428560532397, -289.0518129433099261, -337.3002235550299588 ) ) ;
#9487=CARTESIAN_POINT ( 'NONE',  ( -80.62442908483677684, -283.8240825678217902, -329.2084055579150004 ) ) ;
#9490=CARTESIAN_POINT ( 'NONE',  ( 35.50983018896830856, -295.1469322956708652, -249.5062068842898668 ) ) ;
#9492=CARTESIAN_POINT ( 'NONE',  ( -8.589013747690593448, -293.3685946375959475, -341.3156187562711352 ) ) ;
#9493=CARTESIAN_POINT ( 'NONE',  ( -74.14184375902216573, -276.6129697035595996, -333.6790291688340631 ) ) ;
#9494=CARTESIAN_POINT ( 'NONE',  ( -105.1597938471894622, -296.3710902508544223, -233.9987829939236121 ) ) ;
#9495=CARTESIAN_POINT ( 'NONE',  ( 34.11364144979955881, -292.2676591057815472, -288.3844893160392644 ) ) ;
#9496=CARTESIAN_POINT ( 'NONE',  ( -96.07977523306759338, -295.4171107106524801, -225.3092351886646725 ) ) ;
#9497=CARTESIAN_POINT ( 'NONE',  ( -70.41329951488975780, -292.8111405176712765, -204.8370779666246335 ) ) ;
#9498=CARTESIAN_POINT ( 'NONE',  ( 26.49700095824392321, -294.1393480828650127, -234.2179915113005393 ) ) ;
#9501=CARTESIAN_POINT ( 'NONE',  ( -68.78479238207643220, -293.4643346603442637, -338.6493661170446217 ) ) ;
#9502=CARTESIAN_POINT ( 'NONE',  ( -28.90822910419799285, -300.1578788866440846, -195.3582340379268487 ) ) ;
#9503=CARTESIAN_POINT ( 'NONE',  ( 34.75543000370136326, -288.6625238938570988, -283.2223883440931331 ) ) ;
#9506=CARTESIAN_POINT ( 'NONE',  ( 18.67184088299908140, -278.2313260657311957, -320.7876779903811553 ) ) ;
#9507=CARTESIAN_POINT ( 'NONE',  ( -91.06157840015363547, -276.5893136465502380, -325.0447860595913880 ) ) ;
#9508=CARTESIAN_POINT ( 'NONE',  ( -99.47977570931168145, -272.5038024858304198, -224.9719255903343935 ) ) ;
#9509=CARTESIAN_POINT ( 'NONE',  ( 34.71128871121850068, -279.8746842424320107, -289.1115847744714529 ) ) ;
#9510=CARTESIAN_POINT ( 'NONE',  ( -45.58355504442788941, -275.5546819062440704, -346.1665942128354914 ) ) ;
#9512=CARTESIAN_POINT ( 'NONE',  ( -73.55992231105126677, -294.2284233043565678, -334.3101903791263680 ) ) ;
#9514=CARTESIAN_POINT ( 'NONE',  ( -64.61450876430727419, -274.3378719868794064, -202.5236804764352030 ) ) ;
#9516=CARTESIAN_POINT ( 'NONE',  ( -96.16348885126021173, -289.2169844236783547, -223.2611818973692266 ) ) ;
#9517=CARTESIAN_POINT ( 'NONE',  ( 27.86223874192444683, -274.9399759604181668, -237.5366399163407891 ) ) ;
#9518=CARTESIAN_POINT ( 'NONE',  ( -103.7984261479585228, -290.0447901394413748, -309.3574989870229501 ) ) ;
#9519=CARTESIAN_POINT ( 'NONE',  ( -112.0435739941657403, -274.6592404272614090, -262.0149532151006611 ) ) ;
#9520=CARTESIAN_POINT ( 'NONE',  ( -101.7572472965752013, -294.0403003499689021, -308.5508139450483895 ) ) ;
#9522=CARTESIAN_POINT ( 'NONE',  ( -93.32091865446615486, -283.0292447186187133, -323.0158156954145170 ) ) ;
#9523=ADVANCED_FACE ( 'NONE', ( #69776 ), #47343, .T. ) ;
#9525=CARTESIAN_POINT ( 'NONE',  ( 35.94179950145240809, -279.7576011828080027, -286.3742222304793472 ) ) ;
#9528=CARTESIAN_POINT ( 'NONE',  ( -75.17117814374545048, -290.3311724257180231, -207.4045619966211973 ) ) ;
#9529=CARTESIAN_POINT ( 'NONE',  ( -43.05116421143137018, -281.2644270251465173, -344.4273711321836231 ) ) ;
#9532=CARTESIAN_POINT ( 'NONE',  ( -95.83515293023801007, -289.1979716293355978, -223.3990880863079553 ) ) ;
#9533=CARTESIAN_POINT ( 'NONE',  ( -27.21386722455003593, -275.7031927505482258, -197.3156636692561676 ) ) ;
#9534=CARTESIAN_POINT ( 'NONE',  ( -69.00822795820450040, -284.6644545443642755, -340.1267266683782395 ) ) ;
#9535=CARTESIAN_POINT ( 'NONE',  ( -34.13928655502773069, -272.1719845320087074, -194.8690074849444898 ) ) ;
#9536=CARTESIAN_POINT ( 'NONE',  ( -100.9913200069670296, -285.0424895279036832, -234.5122320193257792 ) ) ;
#9537=CARTESIAN_POINT ( 'NONE',  ( 20.49675419209061644, -277.6142700564980714, -315.8796384092860876 ) ) ;
#9538=CARTESIAN_POINT ( 'NONE',  ( -68.09601417438385340, -278.2694544743675920, -336.7584312091295260 ) ) ;
#9539=CARTESIAN_POINT ( 'NONE',  ( -107.1758150725308241, -286.9099069766326693, -242.8665648304010460 ) ) ;
#9542=CARTESIAN_POINT ( 'NONE',  ( -93.69091745377926372, -295.6699649583649148, -322.8568726151731312 ) ) ;
#9543=CARTESIAN_POINT ( 'NONE',  ( -10.17431246740073902, -288.3884020661536738, -200.8218995084926632 ) ) ;
#9545=CARTESIAN_POINT ( 'NONE',  ( -72.08107566293803359, -286.9809262143061233, -342.4248175857292154 ) ) ;
#9546=CARTESIAN_POINT ( 'NONE',  ( -112.7641495822103792, -277.2971579571951111, -284.3238613800242547 ) ) ;
#9547=CARTESIAN_POINT ( 'NONE',  ( -2.404286826974449287, -290.9063848176224951, -202.6278273392493361 ) ) ;
#9548=CARTESIAN_POINT ( 'NONE',  ( -84.10261485729554920, -286.9162846033334517, -213.3375839668977392 ) ) ;
#9549=CARTESIAN_POINT ( 'NONE',  ( -38.39042639563859893, -281.7989750584970920, -196.3426382076160905 ) ) ;
#9550=CARTESIAN_POINT ( 'NONE',  ( -7.589438515866753221, -287.8597349408465789, -199.9244425422143934 ) ) ;
#9551=CARTESIAN_POINT ( 'NONE',  ( -23.67677284669430904, -284.8776729323631116, -344.1057476738113792 ) ) ;
#9552=CARTESIAN_POINT ( 'NONE',  ( 18.90466005522554127, -276.4360532191820994, -322.9476844291065731 ) ) ;
#9553=CARTESIAN_POINT ( 'NONE',  ( -97.40924347634015135, -295.1799316593315439, -226.0254753265287206 ) ) ;
#9554=CARTESIAN_POINT ( 'NONE',  ( -104.7925647195064727, -278.8665227833717495, -233.2211008802947561 ) ) ;
#9556=CARTESIAN_POINT ( 'NONE',  ( -34.43343589471964350, -300.0089847519888622, -195.9201493502285985 ) ) ;
#9559=CARTESIAN_POINT ( 'NONE',  ( -113.3283667958448859, -270.7922942169334988, -270.3387572857972145 ) ) ;
#9561=CARTESIAN_POINT ( 'NONE',  ( -108.5476548306190523, -277.8434185245061485, -286.7781366562203402 ) ) ;
#9563=CARTESIAN_POINT ( 'NONE',  ( -55.25572410665161982, -275.0317299028056937, -195.8822856719018546 ) ) ;
#9564=CARTESIAN_POINT ( 'NONE',  ( -1.753895159114033486, -281.6510032957936005, -338.3782360564489409 ) ) ;
#9565=CARTESIAN_POINT ( 'NONE',  ( -72.82525072372939690, -291.2891930513913508, -335.3141136941061404 ) ) ;
#9566=CARTESIAN_POINT ( 'NONE',  ( -48.88439730649810855, -299.4279394921284165, -194.8793321862684138 ) ) ;
#9567=CARTESIAN_POINT ( 'NONE',  ( -95.27111034232653708, -297.0765878341701978, -320.4828912119334632 ) ) ;
#9568=CARTESIAN_POINT ( 'NONE',  ( 22.44349852126331868, -294.9357139585002869, -225.3526915261700196 ) ) ;
#9569=CARTESIAN_POINT ( 'NONE',  ( 8.907515791671118066, -280.4163668843435175, -329.2578714169447380 ) ) ;
#9570=CIRCLE ( 'NONE', #62537, 1.897123461337413275 ) ;
#9571=CARTESIAN_POINT ( 'NONE',  ( -24.65454250923442103, -282.1354596386078128, -197.0102473204980242 ) ) ;
#9572=CARTESIAN_POINT ( 'NONE',  ( -78.28397095592997346, -295.5769831587709291, -208.1297061412503240 ) ) ;
#9573=CARTESIAN_POINT ( 'NONE',  ( -109.9173159969080587, -285.8567699480836382, -293.6252306047210823 ) ) ;
#9574=CARTESIAN_POINT ( 'NONE',  ( 12.35529499789633867, -287.2611780074056469, -324.3228928726314280 ) ) ;
#9575=CARTESIAN_POINT ( 'NONE',  ( -102.7707769666400281, -256.8657757996624582, -326.5951631694345565 ) ) ;
#9577=CARTESIAN_POINT ( 'NONE',  ( -40.33399641314547779, -287.6637787920037681, -346.7262601866163436 ) ) ;
#9578=CARTESIAN_POINT ( 'NONE',  ( 28.83090566339503269, -286.8020831496699543, -239.4859867367827917 ) ) ;
#9580=CARTESIAN_POINT ( 'NONE',  ( -76.58784257588565936, -284.6436472105988855, -336.3107154012035949 ) ) ;
#9582=CARTESIAN_POINT ( 'NONE',  ( 33.85342694397820651, -275.6707604746904963, -254.0774322510782497 ) ) ;
#9583=CARTESIAN_POINT ( 'NONE',  ( -27.87356325090788900, -291.0898816066291488, -194.2034736890373097 ) ) ;
#9584=CARTESIAN_POINT ( 'NONE',  ( 36.49951349824269897, -281.9334795679911849, -248.8479575381061863 ) ) ;
#9585=CARTESIAN_POINT ( 'NONE',  ( 21.42425918968850596, -282.4119547273760418, -221.6859725747800098 ) ) ;
#9586=CARTESIAN_POINT ( 'NONE',  ( 17.20513261849135489, -281.1375432829694887, -215.9689100848758017 ) ) ;
#9587=CARTESIAN_POINT ( 'NONE',  ( -9.247346698079034866, -280.4299762035796562, -202.9837678910780880 ) ) ;
#9588=CARTESIAN_POINT ( 'NONE',  ( -37.37352853689063181, -292.5523547857346784, -340.3611179825599606 ) ) ;
#9589=CARTESIAN_POINT ( 'NONE',  ( 122.1772289462398788, 149.4124950158447973, -263.6923987309557447 ) ) ;
#9591=CARTESIAN_POINT ( 'NONE',  ( 33.79687352975842884, -277.2497541240991268, -246.9710812992753972 ) ) ;
#9592=CARTESIAN_POINT ( 'NONE',  ( -31.94682571628636225, -123.9324301101092090, -363.8327245793788620 ) ) ;
#9594=CARTESIAN_POINT ( 'NONE',  ( -65.96931166538414004, -281.4486690165381333, -339.3120012551716513 ) ) ;
#9595=CARTESIAN_POINT ( 'NONE',  ( -106.8010399994768846, -296.2046685995755411, -247.4127002469209913 ) ) ;
#9596=CARTESIAN_POINT ( 'NONE',  ( 13.24273499658139563, -292.2452640551445597, -212.3892124921750337 ) ) ;
#9597=CARTESIAN_POINT ( 'NONE',  ( 180.2407988376923242, 251.0076156727935484, -164.4202208545905535 ) ) ;
#9598=CARTESIAN_POINT ( 'NONE',  ( -15.00602699531519946, -296.9013540461178877, -193.9556305505829812 ) ) ;
#9599=CARTESIAN_POINT ( 'NONE',  ( -105.8633389802770637, -288.5875474646359180, -297.9068605740301905 ) ) ;
#9600=CARTESIAN_POINT ( 'NONE',  ( -2.544137217372268278, -296.4471605080928498, -335.9354658466741625 ) ) ;
#9601=CARTESIAN_POINT ( 'NONE',  ( 4.995878742864167776, -287.9526293940747337, -210.2257885732047384 ) ) ;
#9603=CARTESIAN_POINT ( 'NONE',  ( 39.37218390606714991, -294.5284385272452141, -273.1540033555661466 ) ) ;
#9604=CARTESIAN_POINT ( 'NONE',  ( -108.4268429839573002, -285.2676277954465149, -253.4285056921538057 ) ) ;
#9605=CARTESIAN_POINT ( 'NONE',  ( -82.72293255170497162, -296.2424162609503924, -208.5817507381792097 ) ) ;
#9607=CARTESIAN_POINT ( 'NONE',  ( 15.32003981088454303, -293.5760444376549572, -214.3336259263829504 ) ) ;
#9608=CARTESIAN_POINT ( 'NONE',  ( 39.16423400484711692, -293.9364249304986174, -261.7265915748383804 ) ) ;
#9609=CARTESIAN_POINT ( 'NONE',  ( -82.54460461646614533, -289.8564400820790183, -327.6821213783204598 ) ) ;
#9612=CARTESIAN_POINT ( 'NONE',  ( -23.66215476692705266, -300.0820794693608491, -194.5920294635623691 ) ) ;
#9613=CARTESIAN_POINT ( 'NONE',  ( -63.40748561418260465, -272.5148295702056203, -198.3292948402741160 ) ) ;
#9614=CARTESIAN_POINT ( 'NONE',  ( 21.99556429462856499, -281.2097165398878360, -313.3069080113020277 ) ) ;
#9617=CARTESIAN_POINT ( 'NONE',  ( -95.16868428462585427, -277.3724968870231464, -321.1111604131556305 ) ) ;
#9618=CARTESIAN_POINT ( 'NONE',  ( -87.86631430535015852, -271.7319292938724971, -216.4980116749645163 ) ) ;
#9619=CARTESIAN_POINT ( 'NONE',  ( -109.8177735249234956, -280.6216546491324948, -254.2378388582386890 ) ) ;
#9620=CARTESIAN_POINT ( 'NONE',  ( -62.22582171728111433, -275.5186783481403836, -340.3560777830685424 ) ) ;
#9621=CARTESIAN_POINT ( 'NONE',  ( -90.34317137244825346, -298.4866376724843917, -219.5146078483751637 ) ) ;
#9622=CARTESIAN_POINT ( 'NONE',  ( -94.80476720963775961, -274.1320257151780879, -224.9584267569736937 ) ) ;
#9623=CARTESIAN_POINT ( 'NONE',  ( -113.3291995039209610, -274.3478717295945444, -267.5537497277130683 ) ) ;
#9624=CARTESIAN_POINT ( 'NONE',  ( -0.8200461576269352237, -272.5547160917676024, -204.4330481359575913 ) ) ;
#9625=CARTESIAN_POINT ( 'NONE',  ( 29.58670639534934566, -294.5985647998004993, -299.7631768915263706 ) ) ;
#9626=CARTESIAN_POINT ( 'NONE',  ( -2.141750492084252500, -291.1024768445341238, -205.7222101552331139 ) ) ;
#9628=CARTESIAN_POINT ( 'NONE',  ( 12.66937557499071865, -276.8685166163006102, -328.8283670206632223 ) ) ;
#9629=CARTESIAN_POINT ( 'NONE',  ( 27.86033449979522914, -275.2732823938303000, -237.5328575219699303 ) ) ;
#9630=CARTESIAN_POINT ( 'NONE',  ( -94.04498570814091352, -282.5346182343785131, -321.7423648691323592 ) ) ;
#9631=CARTESIAN_POINT ( 'NONE',  ( 36.28021853227310345, -295.7465373113632268, -285.5216431374584545 ) ) ;
#9633=CARTESIAN_POINT ( 'NONE',  ( -94.24118806243090773, -284.3985009912003648, -224.3515934724798626 ) ) ;
#9634=CARTESIAN_POINT ( 'NONE',  ( -44.27607357025885904, -281.1393677264312032, -345.2593338798153582 ) ) ;
#9636=CARTESIAN_POINT ( 'NONE',  ( 28.39572249904824019, -273.6815862500943695, -237.2859583943369444 ) ) ;
#9637=CARTESIAN_POINT ( 'NONE',  ( 28.84179041037316082, -284.0215787747085869, -305.7508026366863305 ) ) ;
#9638=CARTESIAN_POINT ( 'NONE',  ( 31.64018965405740502, -277.0912415470053816, -295.5813785493502905 ) ) ;
#9641=CARTESIAN_POINT ( 'NONE',  ( -85.28888665664459268, -271.8020784740338627, -211.1369023491587598 ) ) ;
#9643=CARTESIAN_POINT ( 'NONE',  ( -110.6202909622703459, -280.7667899159553144, -253.6196557692183546 ) ) ;
#9646=CARTESIAN_POINT ( 'NONE',  ( 20.96312752533805934, -288.8142182511105602, -222.3001018252047913 ) ) ;
#9649=CARTESIAN_POINT ( 'NONE',  ( -76.62360297572647028, -289.5267465033693952, -206.4115730585729409 ) ) ;
#9651=CARTESIAN_POINT ( 'NONE',  ( -108.9827760595227204, -295.1376887373888280, -286.3200260151753582 ) ) ;
#9652=CARTESIAN_POINT ( 'NONE',  ( 10.90028209779220880, -286.5165004939282767, -326.8522606881854813 ) ) ;
#9653=CARTESIAN_POINT ( 'NONE',  ( 134.9260051231060800, 178.6636279401649858, -236.0341445084446548 ) ) ;
#9655=CARTESIAN_POINT ( 'NONE',  ( 35.28189445654910372, -286.3292427795454955, -293.7816487635085423 ) ) ;
#9656=CARTESIAN_POINT ( 'NONE',  ( -31.73373715014760066, -281.2221778240656249, -346.1536594611444571 ) ) ;
#9657=CARTESIAN_POINT ( 'NONE',  ( -109.7001197232018086, -290.6844909527291634, -260.3291148907240427 ) ) ;
#9660=CARTESIAN_POINT ( 'NONE',  ( 22.30006093257002320, -283.5758584552910975, -313.4899532973534519 ) ) ;
#9661=CARTESIAN_POINT ( 'NONE',  ( 31.51002955751323853, -282.6855108344136056, -295.2504299291638290 ) ) ;
#9662=CARTESIAN_POINT ( 'NONE',  ( -84.12339619002325719, -291.6710849824654588, -329.5028801870471398 ) ) ;
#9663=CARTESIAN_POINT ( 'NONE',  ( -104.2132673289376328, -273.3820114902280807, -232.1235974607446053 ) ) ;
#9665=CARTESIAN_POINT ( 'NONE',  ( -68.78087493636886052, -287.5420300542889436, -339.0840255363177675 ) ) ;
#9666=CARTESIAN_POINT ( 'NONE',  ( 9.510340858009232790, -274.6766464873756490, -209.2555842279344347 ) ) ;
#9667=CARTESIAN_POINT ( 'NONE',  ( -1.675214451139585670, -294.5070912195915298, -204.7741367537638837 ) ) ;
#9669=CARTESIAN_POINT ( 'NONE',  ( -85.33152481854864391, -287.9090924074130839, -210.2361428286349110 ) ) ;
#9670=CARTESIAN_POINT ( 'NONE',  ( -37.15765503423568106, -275.0496619208087736, -345.5403109653299794 ) ) ;
#9672=CARTESIAN_POINT ( 'NONE',  ( -84.70309758908993558, -295.8115657042626481, -210.6674127538477137 ) ) ;
#9673=CARTESIAN_POINT ( 'NONE',  ( -110.7708891840191967, -292.2487011182695369, -262.9723015143296720 ) ) ;
#9674=CARTESIAN_POINT ( 'NONE',  ( -40.77143143020767013, -273.3565983371993298, -197.2899150103065153 ) ) ;
#9675=CARTESIAN_POINT ( 'NONE',  ( -106.6784313101480421, -291.7429396202433054, -295.3235990421428028 ) ) ;
#9677=CARTESIAN_POINT ( 'NONE',  ( -47.03744230239777124, -292.8672274803445816, -197.7704778735459001 ) ) ;
#9678=CARTESIAN_POINT ( 'NONE',  ( -95.90467839396086447, -285.6835378491161350, -315.6405171358399571 ) ) ;
#9679=CARTESIAN_POINT ( 'NONE',  ( -83.92163728383285104, -292.8520801888985261, -209.7228447386410721 ) ) ;
#9680=CARTESIAN_POINT ( 'NONE',  ( -96.21021476626545166, -292.5287890275836844, -221.4757845979581532 ) ) ;
#9681=CARTESIAN_POINT ( 'NONE',  ( 35.20667710874763401, -293.4982800520415935, -278.9126461052029526 ) ) ;
#9682=CARTESIAN_POINT ( 'NONE',  ( 35.01810479133706622, -289.8081786559753255, -290.2786723915117477 ) ) ;
#9683=CARTESIAN_POINT ( 'NONE',  ( 19.78493743910090430, -282.4205870152138687, -322.0680666349201147 ) ) ;
#9684=CARTESIAN_POINT ( 'NONE',  ( -29.22743638579740377, -296.2328265389438684, -194.8037401712774113 ) ) ;
#9685=CARTESIAN_POINT ( 'NONE',  ( -97.57907372424848802, -285.0276190402675525, -222.3980193881760101 ) ) ;
#9686=CARTESIAN_POINT ( 'NONE',  ( 30.57229365799015497, -277.1221266620555070, -239.2597902487837018 ) ) ;
#9687=CARTESIAN_POINT ( 'NONE',  ( -110.4927588826779896, -283.2682903735683908, -276.3655419500586845 ) ) ;
#9688=CARTESIAN_POINT ( 'NONE',  ( 18.80684608830102533, -284.8598328251433713, -220.5617770117214036 ) ) ;
#9689=CARTESIAN_POINT ( 'NONE',  ( -112.8502645824861332, -276.6048669289613713, -277.1956951455856597 ) ) ;
#9691=CARTESIAN_POINT ( 'NONE',  ( -13.51521690613310867, -282.2420721763609777, -339.4820312254543069 ) ) ;
#9692=CARTESIAN_POINT ( 'NONE',  ( -90.79215903166142709, -280.5197032940744180, -215.4140538910143050 ) ) ;
#9693=CARTESIAN_POINT ( 'NONE',  ( 25.65173673949179545, -287.1934814764543944, -314.3231674453072060 ) ) ;
#9694=CARTESIAN_POINT ( 'NONE',  ( 10.96967698473418196, -296.1328630804842419, -326.4323659849628712 ) ) ;
#9695=CARTESIAN_POINT ( 'NONE',  ( -1.822379850096921050, -278.1896645024045256, -337.7763855712681789 ) ) ;
#9696=CARTESIAN_POINT ( 'NONE',  ( -82.24323739268915290, -278.9659198923695271, -332.3058532132864116 ) ) ;
#9697=CARTESIAN_POINT ( 'NONE',  ( -66.80460821013873840, -277.2826198268955977, -337.1513646647946416 ) ) ;
#9698=CARTESIAN_POINT ( 'NONE',  ( 54.45717190063074042, -301.2040501375654458, -195.4963978399819666 ) ) ;
#9699=CARTESIAN_POINT ( 'NONE',  ( 1.132567318379380295, -284.5664680352114715, -206.1153447585900551 ) ) ;
#9700=CARTESIAN_POINT ( 'NONE',  ( -113.5690871964362998, -292.1771159278787877, -268.3958913118173655 ) ) ;
#9701=CARTESIAN_POINT ( 'NONE',  ( -23.47377997482075074, -293.7911545718362163, -342.3984021109696414 ) ) ;
#9703=CARTESIAN_POINT ( 'NONE',  ( -44.29799553449681326, -291.6286053763753330, -197.6212392608824473 ) ) ;
#9705=CARTESIAN_POINT ( 'NONE',  ( -40.31296186643939450, -290.1683176475759751, -347.0074567454298062 ) ) ;
#9706=CARTESIAN_POINT ( 'NONE',  ( -62.35160674059837049, -280.3695924750994095, -201.6170928565556437 ) ) ;
#9707=CARTESIAN_POINT ( 'NONE',  ( -100.4883037576032052, -296.0496371898498182, -226.8179472181121525 ) ) ;
#9708=CARTESIAN_POINT ( 'NONE',  ( 39.53796266087696409, -288.1824963986957187, -268.6787875364595379 ) ) ;
#9709=CARTESIAN_POINT ( 'NONE',  ( 18.63235654641265526, -288.6072984260324006, -323.2066406965383294 ) ) ;
#9710=CARTESIAN_POINT ( 'NONE',  ( -82.80457111999362496, -284.0266621948856027, -327.5680566504572653 ) ) ;
#9711=CARTESIAN_POINT ( 'NONE',  ( -110.4262895430625235, -266.6388475384601406, -306.9518243255819812 ) ) ;
#9713=CARTESIAN_POINT ( 'NONE',  ( -72.24340455811125139, -195.2487258463710589, -358.8499853455330708 ) ) ;
#9714=CARTESIAN_POINT ( 'NONE',  ( -102.6165336565486541, -253.8500844666206717, -324.0719648433210409 ) ) ;
#9715=CARTESIAN_POINT ( 'NONE',  ( -97.02333222867909512, -277.1594937821095073, -312.6995964369357353 ) ) ;
#9716=CARTESIAN_POINT ( 'NONE',  ( -45.95801919408835801, -276.0841584091795085, -343.2129552043403464 ) ) ;
#9717=CARTESIAN_POINT ( 'NONE',  ( -35.82335762372186139, -297.5783404797697926, -193.4227788670093275 ) ) ;
#9718=CARTESIAN_POINT ( 'NONE',  ( 122.9258408653956991, 147.2208392559248296, -261.0359777952371019 ) ) ;
#9719=CARTESIAN_POINT ( 'NONE',  ( -59.53803955172939766, -276.0185769589936058, -343.5773783888014918 ) ) ;
#9722=CARTESIAN_POINT ( 'NONE',  ( -109.2383596609985972, -290.8732257106869383, -283.3556856857578623 ) ) ;
#9723=CARTESIAN_POINT ( 'NONE',  ( -30.51270251543930456, -298.9384395258788913, -193.5216892424431876 ) ) ;
#9724=CARTESIAN_POINT ( 'NONE',  ( 35.24365826826731762, -286.3889136012417680, -281.9568113050851821 ) ) ;
#9725=CARTESIAN_POINT ( 'NONE',  ( -23.37999692633991700, -298.7149106595792887, -193.4215241743794991 ) ) ;
#9726=CARTESIAN_POINT ( 'NONE',  ( -88.50033490900717936, -295.9604296249843856, -322.5070443184440592 ) ) ;
#9729=CIRCLE ( 'NONE', #42998, 5.654241149514405151 ) ;
#9731=CARTESIAN_POINT ( 'NONE',  ( -51.02735006416685337, -279.1458987424568363, -344.6713943997652336 ) ) ;
#9732=CARTESIAN_POINT ( 'NONE',  ( 36.41788400524419700, -281.3367010969636794, -292.4315722113687457 ) ) ;
#9734=CARTESIAN_POINT ( 'NONE',  ( -106.5514983162812968, -279.3098327798778655, -294.6858358276443823 ) ) ;
#9735=CARTESIAN_POINT ( 'NONE',  ( -107.5845723957051376, -280.6855329966974182, -241.3798670223202123 ) ) ;
#9736=CARTESIAN_POINT ( 'NONE',  ( -33.75803411021154687, -296.6726007387902655, -196.7727745394008139 ) ) ;
#9738=CARTESIAN_POINT ( 'NONE',  ( 19.67468459943277992, -281.0747940208947284, -224.7745862308991889 ) ) ;
#9739=CARTESIAN_POINT ( 'NONE',  ( -3.905633187153184416, -275.2848279538511633, -201.1643582922885116 ) ) ;
#9741=CARTESIAN_POINT ( 'NONE',  ( -13.71725678742743781, -276.3589537357258337, -199.1790533596775958 ) ) ;
#9742=CARTESIAN_POINT ( 'NONE',  ( 32.47398523807097348, -274.5263043586089111, -301.4155277852229347 ) ) ;
#9743=ORIENTED_EDGE ( 'NONE', *, *, #57401, .T. ) ;
#9745=CARTESIAN_POINT ( 'NONE',  ( -83.92400360699230077, -290.5900684568355246, -213.9457767266160602 ) ) ;
#9746=CARTESIAN_POINT ( 'NONE',  ( -113.3853541599517030, -284.0482895119258728, -258.5789019710456387 ) ) ;
#9748=CARTESIAN_POINT ( 'NONE',  ( 34.44383347964154041, -279.5568131191429870, -252.2870437996168107 ) ) ;
#9749=CARTESIAN_POINT ( 'NONE',  ( 5.279068719812944011, -279.2163240380427851, -210.3707439335192078 ) ) ;
#9750=CARTESIAN_POINT ( 'NONE',  ( -69.37283355358874815, -283.7072063281451051, -203.1509231710868733 ) ) ;
#9751=CARTESIAN_POINT ( 'NONE',  ( 31.77609534240992417, -289.9341811840557739, -299.6089987112021049 ) ) ;
#9752=CARTESIAN_POINT ( 'NONE',  ( 7.372140313387451016, -281.8820973033118662, -212.0919861584098669 ) ) ;
#9754=CARTESIAN_POINT ( 'NONE',  ( -71.39965445627603913, -281.8942926984311157, -338.5263302623653203 ) ) ;
#9755=CARTESIAN_POINT ( 'NONE',  ( -6.593732790961580825, -296.6485725985107820, -338.7684506057563567 ) ) ;
#9756=CARTESIAN_POINT ( 'NONE',  ( -53.52254542783733626, -278.0873266681529685, -196.0633866177273035 ) ) ;
#9757=CARTESIAN_POINT ( 'NONE',  ( -111.7800635601057451, -286.4138848816814971, -281.1661910985126269 ) ) ;
#9759=CARTESIAN_POINT ( 'NONE',  ( 3.345148980613364742, -294.5141475197300451, -206.6289105848380814 ) ) ;
#9760=CARTESIAN_POINT ( 'NONE',  ( -29.52975948234265502, -274.9531837361189446, -345.0054695198509194 ) ) ;
#9761=CARTESIAN_POINT ( 'NONE',  ( -65.39761142603670407, -288.6067599024544279, -341.9507278319026113 ) ) ;
#9762=CARTESIAN_POINT ( 'NONE',  ( 31.58273731087751912, -291.6035428158867262, -243.9819152356743643 ) ) ;
#9764=CARTESIAN_POINT ( 'NONE',  ( 33.71473966042284331, -274.4831356230225197, -289.1287988120994328 ) ) ;
#9765=CARTESIAN_POINT ( 'NONE',  ( -105.0731592380539610, -294.2877703324295453, -300.8729624262172138 ) ) ;
#9766=CARTESIAN_POINT ( 'NONE',  ( -56.17592060565986856, -290.6149353201861913, -341.4528586170248445 ) ) ;
#9768=CARTESIAN_POINT ( 'NONE',  ( 27.47376236305100861, -291.4993518334920850, -229.9913528745648250 ) ) ;
#9769=CARTESIAN_POINT ( 'NONE',  ( -16.97039141062375123, -287.9196120952910292, -199.3749794889406814 ) ) ;
#9770=CARTESIAN_POINT ( 'NONE',  ( -88.82164420867685806, -288.0033196463141394, -326.2519881607545926 ) ) ;
#9772=CARTESIAN_POINT ( 'NONE',  ( 22.45988901229327439, -288.3817652812061851, -227.3899815451443942 ) ) ;
#9774=CARTESIAN_POINT ( 'NONE',  ( 19.63451674066463681, -287.7073056923214835, -224.4466923867013861 ) ) ;
#9775=CARTESIAN_POINT ( 'NONE',  ( 3.360558448169713941, -296.4883044739045772, -333.8396993327915538 ) ) ;
#9776=CARTESIAN_POINT ( 'NONE',  ( 7.300011400535150408, -287.8504146969630142, -208.0452830692688053 ) ) ;
#9777=CARTESIAN_POINT ( 'NONE',  ( -99.29902237962620859, -276.0494080346783221, -313.6116025848223785 ) ) ;
#9778=CARTESIAN_POINT ( 'NONE',  ( -113.7447166088730768, -278.7625871955591492, -280.1810138114370261 ) ) ;
#9779=CARTESIAN_POINT ( 'NONE',  ( 10.81308941622893727, -280.3637467699149397, -210.2356486785652976 ) ) ;
#9780=CARTESIAN_POINT ( 'NONE',  ( -53.00427921903821726, -299.8304358388951982, -197.3249770768330507 ) ) ;
#9781=CARTESIAN_POINT ( 'NONE',  ( -40.02052801174312435, -284.0183229268633340, -195.4089696973081232 ) ) ;
#9783=CARTESIAN_POINT ( 'NONE',  ( -79.74127196714272259, -277.6117016336031043, -209.4255636160433482 ) ) ;
#9784=CARTESIAN_POINT ( 'NONE',  ( -60.63534809389868485, -281.3540195771609547, -341.7063627447745944 ) ) ;
#9786=CARTESIAN_POINT ( 'NONE',  ( -34.33794152799971044, -275.4949121717301068, -346.6086437673907312 ) ) ;
#9787=CARTESIAN_POINT ( 'NONE',  ( -96.14599511751498540, -297.4539419530267423, -314.7976917115472588 ) ) ;
#9788=CARTESIAN_POINT ( 'NONE',  ( 23.15058279763064419, -281.1050318346463541, -317.5222990162498036 ) ) ;
#9789=CARTESIAN_POINT ( 'NONE',  ( -109.2790518340333108, -297.6747840242583152, -256.5674410555818667 ) ) ;
#9790=CARTESIAN_POINT ( 'NONE',  ( -111.8218348645858811, -297.6464213469399738, -287.9108098609399917 ) ) ;
#9791=CARTESIAN_POINT ( 'NONE',  ( 22.30055460734150330, -274.6307383756973763, -228.2100405927494933 ) ) ;
#9792=CARTESIAN_POINT ( 'NONE',  ( -11.59696698761547573, -294.3874482099959096, -199.8628208135307318 ) ) ;
#9793=CARTESIAN_POINT ( 'NONE',  ( 14.24530587071075161, -286.9197968553933720, -213.1250789842667075 ) ) ;
#9794=CARTESIAN_POINT ( 'NONE',  ( -39.52076249630715665, -278.1048740695651986, -194.8197344119153342 ) ) ;
#9796=CARTESIAN_POINT ( 'NONE',  ( -112.9245502226013969, -290.5702363738715235, -255.5875854675222456 ) ) ;
#9797=CARTESIAN_POINT ( 'NONE',  ( -105.3359527187882207, -289.2463177848592295, -297.7037137619369105 ) ) ;
#9798=CARTESIAN_POINT ( 'NONE',  ( 18.89634741421465947, -290.8620007685027531, -220.7203140196610605 ) ) ;
#9799=VERTEX_POINT ( 'NONE', #55108 ) ;
#9800=CARTESIAN_POINT ( 'NONE',  ( 185.2614386149834900, 255.8498544563436212, -168.8850006258623466 ) ) ;
#9801=CARTESIAN_POINT ( 'NONE',  ( -34.58195314628625994, -288.5243327706897389, -343.4201401007718459 ) ) ;
#9803=CARTESIAN_POINT ( 'NONE',  ( -112.2927515526778564, -285.2853080173690046, -286.9490685634335705 ) ) ;
#9804=CARTESIAN_POINT ( 'NONE',  ( 23.79513032152149776, -291.9901604993756337, -223.9163402126301037 ) ) ;
#9805=CARTESIAN_POINT ( 'NONE',  ( 26.32087894317058385, -283.4294005228077253, -312.7919357759415107 ) ) ;
#9806=CARTESIAN_POINT ( 'NONE',  ( -104.1141557471359818, -283.9884278403224016, -299.8643241657096041 ) ) ;
#9807=CARTESIAN_POINT ( 'NONE',  ( -97.34634728117254099, -297.1988415976783244, -222.1071821841918847 ) ) ;
#9808=CARTESIAN_POINT ( 'NONE',  ( 17.81636526077367932, -277.5563473228442604, -318.9479098553642871 ) ) ;
#9809=CARTESIAN_POINT ( 'NONE',  ( -63.35073507984012764, -289.7316987517211260, -200.3941478945161521 ) ) ;
#9811=CARTESIAN_POINT ( 'NONE',  ( -48.92304016706964376, -272.6963947151297702, -197.8320633928682355 ) ) ;
#9814=CARTESIAN_POINT ( 'NONE',  ( -84.58018157659009262, -287.3162523268560449, -212.7629163056879236 ) ) ;
#9815=CARTESIAN_POINT ( 'NONE',  ( -94.41231436011754852, -296.9337271715625093, -321.6099434708485205 ) ) ;
#9816=CARTESIAN_POINT ( 'NONE',  ( -110.4923597237573745, -285.1962291497000592, -270.9183435146323973 ) ) ;
#9817=CARTESIAN_POINT ( 'NONE',  ( 8.092125093130805524, -275.5069109236012537, -332.3025060009279628 ) ) ;
#9818=CARTESIAN_POINT ( 'NONE',  ( 8.783148742161767331, -293.3170895263070861, -208.7657199287959031 ) ) ;
#9819=CARTESIAN_POINT ( 'NONE',  ( 25.34885385511638844, -285.1214030380116355, -227.7914877013124055 ) ) ;
#9820=CARTESIAN_POINT ( 'NONE',  ( 39.41966412220719462, -293.8130945796434617, -264.5786228559652500 ) ) ;
#9821=CARTESIAN_POINT ( 'NONE',  ( -108.7321347707435137, -291.0878121699835219, -255.0153261033129581 ) ) ;
#9824=CARTESIAN_POINT ( 'NONE',  ( 6.292094988509354891, -59.58581467011203614, -351.0172641016240505 ) ) ;
#9825=CARTESIAN_POINT ( 'NONE',  ( -113.6342575831652368, -286.1126340743217042, -267.1629504333221803 ) ) ;
#9826=CARTESIAN_POINT ( 'NONE',  ( -2.659677404128736544, -274.1237833571632905, -342.4524372437778652 ) ) ;
#9828=CARTESIAN_POINT ( 'NONE',  ( -109.0252103026800938, -283.2700229538513099, -285.7733293863130939 ) ) ;
#9829=CARTESIAN_POINT ( 'NONE',  ( -112.1556390077946332, -277.9914063238471158, -288.5441879536006127 ) ) ;
#9830=CARTESIAN_POINT ( 'NONE',  ( 36.12945993587742777, -283.3685413907255679, -256.0804567259272062 ) ) ;
#9831=CARTESIAN_POINT ( 'NONE',  ( -97.34057529231125727, -248.7244481610983087, -333.3648534768652780 ) ) ;
#9832=CARTESIAN_POINT ( 'NONE',  ( -83.54149235775581417, -282.2461979953035893, -331.2896159282820463 ) ) ;
#9833=CARTESIAN_POINT ( 'NONE',  ( 34.98849370620082055, -285.3335742626629212, -251.8652202634366688 ) ) ;
#9834=CARTESIAN_POINT ( 'NONE',  ( 25.11272978387250276, -276.8369696826169388, -227.4458297074222060 ) ) ;
#9835=CARTESIAN_POINT ( 'NONE',  ( -20.82817513350164162, -295.3269101086378328, -341.5841320997348021 ) ) ;
#9836=CARTESIAN_POINT ( 'NONE',  ( 4.800036883009760835, -291.3191363122518283, -210.0881147899867187 ) ) ;
#9837=CARTESIAN_POINT ( 'NONE',  ( -96.06597149290826110, -278.5335842364756900, -320.0279166731389751 ) ) ;
#9838=CARTESIAN_POINT ( 'NONE',  ( -27.02151370780244122, -276.9172729085353239, -342.6279412990078868 ) ) ;
#9839=CARTESIAN_POINT ( 'NONE',  ( 19.63828796805541188, -275.1722565129433633, -321.7108111205922114 ) ) ;
#9841=CARTESIAN_POINT ( 'NONE',  ( -37.81293164330911338, -275.0579264444754131, -345.3722021308782359 ) ) ;
#9843=CARTESIAN_POINT ( 'NONE',  ( 3.924473101418306520, -295.9337739410519248, -334.7329023063056184 ) ) ;
#9846=CARTESIAN_POINT ( 'NONE',  ( -89.10284742764287103, -284.8805173293629309, -322.3458382200366827 ) ) ;
#9847=CARTESIAN_POINT ( 'NONE',  ( -33.09270350509498826, -284.7594926595880338, -346.2418599714705465 ) ) ;
#9848=CARTESIAN_POINT ( 'NONE',  ( -10.70511129342985690, -285.7575212949250840, -202.2712564899942151 ) ) ;
#9849=CARTESIAN_POINT ( 'NONE',  ( 28.73783559161208245, -274.3941693347215391, -303.3386281445947361 ) ) ;
#9850=CARTESIAN_POINT ( 'NONE',  ( 35.44641809470454774, -283.6026141821849365, -285.0113242216903018 ) ) ;
#9851=CARTESIAN_POINT ( 'NONE',  ( -109.9726944037626311, -276.8681261896258547, -282.9036337822892619 ) ) ;
#9852=CARTESIAN_POINT ( 'NONE',  ( -21.57318746054862402, -277.9250244664475531, -342.0064894934947688 ) ) ;
#9854=CARTESIAN_POINT ( 'NONE',  ( 35.17189338322290126, -282.0319481775883332, -244.7869617890567895 ) ) ;
#9855=CARTESIAN_POINT ( 'NONE',  ( -38.17553398408971077, -280.5343091141434684, -193.4271747283714262 ) ) ;
#9859=CARTESIAN_POINT ( 'NONE',  ( 36.80964199851275964, -289.2140874069019105, -254.7457740286168644 ) ) ;
#9860=CARTESIAN_POINT ( 'NONE',  ( -77.59230153146845055, -296.6941246685178157, -209.2061314547664495 ) ) ;
#9861=CARTESIAN_POINT ( 'NONE',  ( -84.19766316037826925, -290.7757288606391626, -209.3199886476936342 ) ) ;
#9863=CARTESIAN_POINT ( 'NONE',  ( 34.37136329923080069, -286.2537841291144787, -287.3300392358489717 ) ) ;
#9864=CARTESIAN_POINT ( 'NONE',  ( -26.40510210283736114, -287.4851145156978873, -343.1845903235468427 ) ) ;
#9865=CARTESIAN_POINT ( 'NONE',  ( -9.356116832418225115, -287.6313537156144093, -202.4952158166496190 ) ) ;
#9866=CARTESIAN_POINT ( 'NONE',  ( -95.51957283810780552, -275.8997473858997864, -317.7134222536338370 ) ) ;
#9867=CARTESIAN_POINT ( 'NONE',  ( 35.61350560996478976, -286.2315701808482231, -292.4059039905488362 ) ) ;
#9868=CARTESIAN_POINT ( 'NONE',  ( 36.06071206279163732, -289.3538093307945473, -254.9014189386541318 ) ) ;
#9869=CARTESIAN_POINT ( 'NONE',  ( -54.11782974035947547, -287.2667779930648067, -343.6851928737355593 ) ) ;
#9870=CARTESIAN_POINT ( 'NONE',  ( 25.76786062151803591, -283.0033063016231836, -307.6176703856384620 ) ) ;
#9871=CARTESIAN_POINT ( 'NONE',  ( -111.0647581494525440, -292.3636499960987862, -285.0870527662316363 ) ) ;
#9874=CARTESIAN_POINT ( 'NONE',  ( -94.49818481850003593, -299.1532571841493109, -220.8618432982795525 ) ) ;
#9875=CARTESIAN_POINT ( 'NONE',  ( -32.94311282739938207, -279.3061489930066159, -197.3319857342073078 ) ) ;
#9876=CARTESIAN_POINT ( 'NONE',  ( 34.12965940181446456, -279.8473453391552539, -293.2643087542202807 ) ) ;
#9877=CARTESIAN_POINT ( 'NONE',  ( 36.93784224080613399, -292.9960305013196376, -290.0260208911292921 ) ) ;
#9878=CARTESIAN_POINT ( 'NONE',  ( -83.80962717219931335, -271.6437861450824016, -212.7529087836911117 ) ) ;
#9879=CARTESIAN_POINT ( 'NONE',  ( -10.76227492213332226, -274.7826462363113933, -339.8941917943659519 ) ) ;
#9880=CARTESIAN_POINT ( 'NONE',  ( -99.13895738467218166, -297.3193845195517042, -310.2329832237285814 ) ) ;
#9882=CARTESIAN_POINT ( 'NONE',  ( 18.77375479150365933, -297.2225164868111165, -194.0686380784358391 ) ) ;
#9883=CARTESIAN_POINT ( 'NONE',  ( -74.13560225244695800, -293.7736376000908081, -336.9045079275734338 ) ) ;
#9885=CARTESIAN_POINT ( 'NONE',  ( 23.06128707832070646, -294.3959680663696759, -228.3049597045583141 ) ) ;
#9887=CARTESIAN_POINT ( 'NONE',  ( 26.37015791516194341, -293.8625538294185162, -234.2938191352998274 ) ) ;
#9889=CARTESIAN_POINT ( 'NONE',  ( -33.77931186183484868, -284.1168854587702981, -195.0901661182930695 ) ) ;
#9890=CARTESIAN_POINT ( 'NONE',  ( -47.79303666712760901, -295.1886229446446350, -342.6603706623741346 ) ) ;
#9891=CARTESIAN_POINT ( 'NONE',  ( -50.09350821601505999, -283.2104416505460449, -346.3517522504720318 ) ) ;
#9892=CARTESIAN_POINT ( 'NONE',  ( 22.58992810886332947, -282.8465046359950179, -224.3235344374665203 ) ) ;
#9893=CARTESIAN_POINT ( 'NONE',  ( -109.0072414961743306, -284.5768410370488368, -242.1128923590738395 ) ) ;
#9894=CARTESIAN_POINT ( 'NONE',  ( -112.1705501103153182, -288.5414404816520459, -271.1806506031392701 ) ) ;
#9896=CARTESIAN_POINT ( 'NONE',  ( 25.34956039056106647, -280.6122332085997755, -313.8871202295876515 ) ) ;
#9897=CARTESIAN_POINT ( 'NONE',  ( -10.55472642596464183, -285.0938676076682441, -201.9099254332658404 ) ) ;
#9898=CARTESIAN_POINT ( 'NONE',  ( -4.478041913113405492, -287.5495392352121371, -339.6681960487437664 ) ) ;
#9900=CARTESIAN_POINT ( 'NONE',  ( -12.72236635771002788, -296.3269730412072249, -339.9874377601415176 ) ) ;
#9901=CARTESIAN_POINT ( 'NONE',  ( -86.70062840136722571, -279.1477484668685634, -328.7595926825929382 ) ) ;
#9902=CARTESIAN_POINT ( 'NONE',  ( -14.30927091733863676, -292.7750434281453522, -342.1100831703632821 ) ) ;
#9903=CARTESIAN_POINT ( 'NONE',  ( -68.52847119376930607, -279.2973688576392419, -204.3348141531652686 ) ) ;
#9904=CARTESIAN_POINT ( 'NONE',  ( -2.057729579103245499, -292.6729075361406558, -201.9062833302965601 ) ) ;
#9905=CARTESIAN_POINT ( 'NONE',  ( -109.5426468588345159, -282.9191558380418314, -247.9065675782656228 ) ) ;
#9907=CARTESIAN_POINT ( 'NONE',  ( -48.17914321879006678, -279.1900778574910191, -344.6264829827023277 ) ) ;
#9908=CARTESIAN_POINT ( 'NONE',  ( -3.044139853223456260, -293.6459454442413630, -335.0688131032514434 ) ) ;
#9909=CARTESIAN_POINT ( 'NONE',  ( -67.35312805639196654, -295.6585651308055276, -201.5721544375535927 ) ) ;
#9910=VERTEX_POINT ( 'NONE', #68851 ) ;
#9912=CARTESIAN_POINT ( 'NONE',  ( -11.18999682103091686, -282.3743959738797571, -200.3926948210630599 ) ) ;
#9913=CARTESIAN_POINT ( 'NONE',  ( -110.1611162163360973, -295.9736302621539039, -276.8989164124456579 ) ) ;
#9914=DIRECTION ( 'NONE',  ( 1.000000000000000000, 0.000000000000000000, 0.000000000000000000 ) ) ;
#9915=CARTESIAN_POINT ( 'NONE',  ( -69.85430415644619018, -271.1237833571632905, -202.7746430608542312 ) ) ;
#9916=CARTESIAN_POINT ( 'NONE',  ( -111.6594595240124619, -271.9965132982247269, -250.6376077469666370 ) ) ;
#9917=CARTESIAN_POINT ( 'NONE',  ( 36.89423065911203281, -288.6343510633527103, -251.8590949951244227 ) ) ;
#9918=CARTESIAN_POINT ( 'NONE',  ( -74.71772516099515826, -289.3979432552050639, -333.0817278144757552 ) ) ;
#9919=CARTESIAN_POINT ( 'NONE',  ( -5.274120841319772879, -282.0021661177767669, -204.0106988921551761 ) ) ;
#9920=CARTESIAN_POINT ( 'NONE',  ( -63.45772478805206163, -299.4673947567290497, -201.0542547850966173 ) ) ;
#9921=CARTESIAN_POINT ( 'NONE',  ( -79.26919076345298265, -278.2669363119382524, -210.1181430150086555 ) ) ;
#9923=CARTESIAN_POINT ( 'NONE',  ( -104.2284779812430600, -272.8821307731292336, -232.1075735540319727 ) ) ;
#9924=CARTESIAN_POINT ( 'NONE',  ( -100.9546090670384615, -292.9944419588503024, -231.6996124152321670 ) ) ;
#9926=CARTESIAN_POINT ( 'NONE',  ( -82.60289083594690851, -290.3410952500420876, -327.7659721634676657 ) ) ;
#9928=CARTESIAN_POINT ( 'NONE',  ( 35.11279740381718995, -291.4090784477664329, -248.2104685958580035 ) ) ;
#9929=CARTESIAN_POINT ( 'NONE',  ( -69.26294878366692842, -297.2868899521721460, -204.6867594310858749 ) ) ;
#9931=CARTESIAN_POINT ( 'NONE',  ( -111.8838571220086493, -291.8663737897115880, -286.6759758174366652 ) ) ;
#9932=CARTESIAN_POINT ( 'NONE',  ( 25.18497378105907814, -289.4090924074130839, -220.4570493818173702 ) ) ;
#9933=CARTESIAN_POINT ( 'NONE',  ( 36.33096146400724535, -289.7212613059061823, -283.4899931212314073 ) ) ;
#9934=CARTESIAN_POINT ( 'NONE',  ( 26.93764601780200252, -274.0659118134340133, -308.6781387921165560 ) ) ;
#9935=CARTESIAN_POINT ( 'NONE',  ( 35.52600146347161569, -277.2746245475428850, -255.0801729698249858 ) ) ;
#9936=CARTESIAN_POINT ( 'NONE',  ( 27.50068826931539689, -291.1400055566363676, -233.6938217431761302 ) ) ;
#9937=CARTESIAN_POINT ( 'NONE',  ( -90.21344657196837602, -281.1749379213878797, -216.0211708448780143 ) ) ;
#9939=ORIENTED_EDGE ( 'NONE', *, *, #13746, .F. ) ;
#9940=CARTESIAN_POINT ( 'NONE',  ( -40.24670249014474166, -282.4382147928780569, -343.4053075509805240 ) ) ;
#9941=CARTESIAN_POINT ( 'NONE',  ( -95.90421196187325847, -278.9617731786528907, -319.8982959258485153 ) ) ;
#9942=CARTESIAN_POINT ( 'NONE',  ( -4.348827258955087594, -281.4218677185662614, -339.5093072718176472 ) ) ;
#9943=CARTESIAN_POINT ( 'NONE',  ( -89.04476833809601999, -278.6995507975592545, -327.1027512870687133 ) ) ;
#9946=CARTESIAN_POINT ( 'NONE',  ( -55.19039093520709827, -275.3467254329793263, -196.1712804887263815 ) ) ;
#9947=CARTESIAN_POINT ( 'NONE',  ( -105.5795714935544112, -280.8376638359844151, -285.9686137636504668 ) ) ;
#9949=CARTESIAN_POINT ( 'NONE',  ( -110.7416098782010891, -298.7509451859120304, -254.8897257155112186 ) ) ;
#9950=CARTESIAN_POINT ( 'NONE',  ( -109.7221141836586611, -291.4779942927941647, -282.0719114613131069 ) ) ;
#9951=CARTESIAN_POINT ( 'NONE',  ( -99.03427638254679266, -291.7161585215891932, -314.7455486226522225 ) ) ;
#9952=CARTESIAN_POINT ( 'NONE',  ( -87.99525036370171449, -290.6696676790480751, -217.5833860367995953 ) ) ;
#9953=CARTESIAN_POINT ( 'NONE',  ( 36.63379597003661559, -286.7923764334385055, -249.0258990881542900 ) ) ;
#9955=CARTESIAN_POINT ( 'NONE',  ( -26.64676077994170100, -281.3138494874469870, -343.4339249386031270 ) ) ;
#9956=CARTESIAN_POINT ( 'NONE',  ( -10.25163302473109717, -290.5553476767098005, -339.5320586341034641 ) ) ;
#9957=CARTESIAN_POINT ( 'NONE',  ( -109.1048677774284528, -282.8124165396556009, -287.1720772192215350 ) ) ;
#9958=CARTESIAN_POINT ( 'NONE',  ( -6.578175613760438800, -281.7799452396975539, -203.6027257611767709 ) ) ;
#9959=CARTESIAN_POINT ( 'NONE',  ( -5.712459371392874630, -289.5875332037014687, -340.3068922860259704 ) ) ;
#9960=CARTESIAN_POINT ( 'NONE',  ( -64.84509111272539883, -280.1753177911814987, -202.6739557870255624 ) ) ;
#9961=CARTESIAN_POINT ( 'NONE',  ( 35.08225795746511011, -292.0290671447872342, -245.2449159236358867 ) ) ;
#9962=CARTESIAN_POINT ( 'NONE',  ( 23.72686322068857123, -287.7316625933499381, -223.7049114343797669 ) ) ;
#9963=CARTESIAN_POINT ( 'NONE',  ( 20.23652376549609500, -287.3519379484955039, -219.2503823002382717 ) ) ;
#9964=CARTESIAN_POINT ( 'NONE',  ( -91.66362565694265641, -284.0206987331293931, -319.1459847004953758 ) ) ;
#9967=CARTESIAN_POINT ( 'NONE',  ( 35.09892406273690568, -295.1293097740040139, -248.1651397951241620 ) ) ;
#9968=CARTESIAN_POINT ( 'NONE',  ( 38.73762242568383130, -292.1291950292558681, -261.7978606863005666 ) ) ;
#9969=CARTESIAN_POINT ( 'NONE',  ( -64.43129076525022469, -276.4732150278147174, -338.4558663469026669 ) ) ;
#9970=CARTESIAN_POINT ( 'NONE',  ( -112.7870606520255166, -296.0878875200045854, -255.4169339165041208 ) ) ;
#9971=CARTESIAN_POINT ( 'NONE',  ( 34.89996748549255301, -291.8418287558436646, -255.8060771180843460 ) ) ;
#9972=CARTESIAN_POINT ( 'NONE',  ( -94.38034297048322685, -295.4517127757300159, -223.1760903312505491 ) ) ;
#9973=CARTESIAN_POINT ( 'NONE',  ( -47.06215973795028873, -293.1310087205572472, -197.6105635572535562 ) ) ;
#9974=CARTESIAN_POINT ( 'NONE',  ( 14.54473894379112231, -295.3808295260497516, -322.2207643882104549 ) ) ;
#9976=CARTESIAN_POINT ( 'NONE',  ( -58.36360920679964437, -293.3229525051447695, -342.5825932733167178 ) ) ;
#9977=CARTESIAN_POINT ( 'NONE',  ( -103.6897508074134038, -299.0170822937945445, -235.2808793229553430 ) ) ;
#9978=CARTESIAN_POINT ( 'NONE',  ( 29.01811925908577550, -288.0764112151803147, -239.3807561661215857 ) ) ;
#9979=CARTESIAN_POINT ( 'NONE',  ( 30.38823470957666117, -277.9667574367251746, -303.5112904689913762 ) ) ;
#9980=CARTESIAN_POINT ( 'NONE',  ( -51.25563148528563318, -276.0211720234513564, -345.6898059554854399 ) ) ;
#9981=CARTESIAN_POINT ( 'NONE',  ( -7.722162016759400061, -273.7787423754169254, -199.3398424528018040 ) ) ;
#9982=CARTESIAN_POINT ( 'NONE',  ( 12.87034856786478798, -280.4245380306837205, -325.3162302230959426 ) ) ;
#9983=CARTESIAN_POINT ( 'NONE',  ( 3.059882193921571680, -274.9195427624969170, -335.0309020544182772 ) ) ;
#9984=CARTESIAN_POINT ( 'NONE',  ( -109.7589535603569573, -295.4011480807924386, -257.8317571024118706 ) ) ;
#9985=DIRECTION ( 'NONE',  ( -1.000000000000000000, -0.000000000000000000, -0.000000000000000000 ) ) ;
#9986=CARTESIAN_POINT ( 'NONE',  ( -104.4766043141997187, -273.5932745095020096, -241.3053539905463367 ) ) ;
#9988=CARTESIAN_POINT ( 'NONE',  ( -107.2814458553013424, -288.2085156541588731, -298.4117644639158584 ) ) ;
#9989=CARTESIAN_POINT ( 'NONE',  ( 21.48244090413423280, -274.7798036787380624, -227.1324187615000767 ) ) ;
#9990=CARTESIAN_POINT ( 'NONE',  ( -17.72432682165848306, -288.8058899575905230, -344.8202253137417301 ) ) ;
#9991=CARTESIAN_POINT ( 'NONE',  ( -51.51647858738688512, -299.8517702051267406, -196.2979200959672994 ) ) ;
#9992=CARTESIAN_POINT ( 'NONE',  ( -102.8063700430792125, -295.0353824842449058, -234.1063884039852212 ) ) ;
#9993=CARTESIAN_POINT ( 'NONE',  ( -96.15333330122081179, -283.0818777094344796, -319.8319661097800122 ) ) ;
#9995=CARTESIAN_POINT ( 'NONE',  ( -72.45220931098012329, -281.5166370790795440, -336.6495233384585504 ) ) ;
#9998=CARTESIAN_POINT ( 'NONE',  ( -84.07009452426848384, -290.1878900372651060, -213.7608736298832355 ) ) ;
#9999=CARTESIAN_POINT ( 'NONE',  ( -104.1342104250410330, -282.2590610662592212, -302.8771847243558000 ) ) ;
#10001=DIRECTION ( 'NONE',  ( 0.01273136352371030157, 0.9999189529070979798, 0.000000000000000000 ) ) ;
#10002=CARTESIAN_POINT ( 'NONE',  ( -94.96042251753112851, -289.2152406154886535, -222.3297927940171235 ) ) ;
#10003=CARTESIAN_POINT ( 'NONE',  ( -67.35746438392645530, -275.1713385687233426, -203.0437890354925798 ) ) ;
#10004=CARTESIAN_POINT ( 'NONE',  ( -8.175779688113395949, -283.8837834530419286, -341.2506814278392540 ) ) ;
#10005=CARTESIAN_POINT ( 'NONE',  ( 4.094315903279943214, -272.6851563448075808, -207.1138175289611354 ) ) ;
#10006=CARTESIAN_POINT ( 'NONE',  ( -88.89429033568079319, -283.8010199160273146, -322.1169842834329415 ) ) ;
#10007=CARTESIAN_POINT ( 'NONE',  ( 19.64935706065706711, -277.6314969295889341, -316.9362636418679244 ) ) ;
#10008=CARTESIAN_POINT ( 'NONE',  ( -61.83427240088293075, -278.1814975978680877, -339.3549167273005196 ) ) ;
#10010=CARTESIAN_POINT ( 'NONE',  ( 28.03145067257481315, -284.0431787727699202, -307.2277630360985654 ) ) ;
#10012=PLANE ( 'NONE',  #25591 ) ;
#10013=CARTESIAN_POINT ( 'NONE',  ( -4.504459831131269354, -294.4646721581770521, -340.0226669062264477 ) ) ;
#10014=CARTESIAN_POINT ( 'NONE',  ( -30.40294396809127164, -288.1200987561765032, -195.9875741171783829 ) ) ;
#10015=CARTESIAN_POINT ( 'NONE',  ( 114.7448031289451222, -296.6656502513747569, -195.3611179825600175 ) ) ;
#10016=CARTESIAN_POINT ( 'NONE',  ( -111.2869819898779866, -287.6237833571632905, -305.9350535429201159 ) ) ;
#10017=CARTESIAN_POINT ( 'NONE',  ( -84.36650604195679648, -278.3427919080723996, -209.7120769616728637 ) ) ;
#10018=CARTESIAN_POINT ( 'NONE',  ( -95.95035890381885224, -289.6139582180073830, -221.6432655608323330 ) ) ;
#10019=CARTESIAN_POINT ( 'NONE',  ( -108.4248537068418017, -285.8173032810881296, -289.8481844162884613 ) ) ;
#10020=CARTESIAN_POINT ( 'NONE',  ( -41.89686238152864917, -278.8704480035421511, -344.2469189503393636 ) ) ;
#10021=CARTESIAN_POINT ( 'NONE',  ( 13.83864486679501660, -288.1781864971354707, -213.5523415782789414 ) ) ;
#10022=CARTESIAN_POINT ( 'NONE',  ( 35.60111004784599942, -283.7770093047340652, -287.8613781295371155 ) ) ;
#10023=CARTESIAN_POINT ( 'NONE',  ( 10.52771815065294625, -276.5787318250444287, -330.7410510484766064 ) ) ;
#10024=CARTESIAN_POINT ( 'NONE',  ( -91.21590465307482987, -295.3021833736847270, -218.6207752515046536 ) ) ;
#10025=CARTESIAN_POINT ( 'NONE',  ( -98.57506698344418794, -279.0080531743761867, -223.6547949431706854 ) ) ;
#10026=CARTESIAN_POINT ( 'NONE',  ( -67.42323911292918126, -299.5746791046591966, -202.2559387275920244 ) ) ;
#10029=CARTESIAN_POINT ( 'NONE',  ( -94.62145573745037552, -295.3732980830532711, -220.6911650413244388 ) ) ;
#10031=CARTESIAN_POINT ( 'NONE',  ( -99.23055486891736621, -277.5229251376787829, -309.2854930727917235 ) ) ;
#10032=CARTESIAN_POINT ( 'NONE',  ( 13.68846862446016743, -275.9532887817881601, -213.1594267440934800 ) ) ;
#10033=CARTESIAN_POINT ( 'NONE',  ( 39.47505563341835710, -280.6056632643965258, -269.9435485344857852 ) ) ;
#10034=CARTESIAN_POINT ( 'NONE',  ( -34.51718406982833187, -290.7764571392863218, -344.3708089446921576 ) ) ;
#10035=CARTESIAN_POINT ( 'NONE',  ( -106.5295068657478481, -297.6566176777852206, -302.5442680727112474 ) ) ;
#10036=CARTESIAN_POINT ( 'NONE',  ( -76.86414466607730844, -296.7737164462395185, -336.0428272258292850 ) ) ;
#10037=CARTESIAN_POINT ( 'NONE',  ( 34.37900947287858600, -295.2744938955358975, -248.8246693847556514 ) ) ;
#10038=CARTESIAN_POINT ( 'NONE',  ( 31.72305642217235899, -279.1749930202285555, -241.5498731901628275 ) ) ;
#10039=CARTESIAN_POINT ( 'NONE',  ( -46.66050028238030478, -281.8532458216003533, -196.4545942326763281 ) ) ;
#10040=CARTESIAN_POINT ( 'NONE',  ( -107.1478338048257513, -294.9718139683891422, -244.3587901969843585 ) ) ;
#10041=CARTESIAN_POINT ( 'NONE',  ( -99.12771944298239646, -285.5536982517733122, -315.0466683873710849 ) ) ;
#10042=CARTESIAN_POINT ( 'NONE',  ( 23.79944016464181189, -285.9125904452710643, -229.8218499948106626 ) ) ;
#10043=CARTESIAN_POINT ( 'NONE',  ( 39.60848648064015265, -280.8954554044021847, -269.9391182948613164 ) ) ;
#10044=CARTESIAN_POINT ( 'NONE',  ( 175.7043253900435786, 241.9494694207491534, -179.2918632058347157 ) ) ;
#10046=CARTESIAN_POINT ( 'NONE',  ( -29.05922573830736511, -287.5240033711278329, -346.3747949725814692 ) ) ;
#10047=CARTESIAN_POINT ( 'NONE',  ( 4.741015212186894701, -286.3044395497469168, -210.6240142159401216 ) ) ;
#10049=CARTESIAN_POINT ( 'NONE',  ( -55.61515296490964744, -284.3616968247805517, -344.8431522612921185 ) ) ;
#10050=CARTESIAN_POINT ( 'NONE',  ( 32.08059082321670274, -275.5831436183505048, -247.5570882805398014 ) ) ;
#10051=CARTESIAN_POINT ( 'NONE',  ( -74.51697224360025018, -290.4898246469914511, -203.2828677576506209 ) ) ;
#10052=CARTESIAN_POINT ( 'NONE',  ( 39.53837978329480762, -282.1621426936807779, -267.0534761568782187 ) ) ;
#10054=CARTESIAN_POINT ( 'NONE',  ( -111.0662224004974377, -280.3215223886096510, -250.6280784346119219 ) ) ;
#10055=CARTESIAN_POINT ( 'NONE',  ( 23.72793881191635279, -281.2598884821137517, -223.4754897898779973 ) ) ;
#10056=CARTESIAN_POINT ( 'NONE',  ( 27.33386217378598815, -285.4809262143061801, -301.5434626090942629 ) ) ;
#10057=CARTESIAN_POINT ( 'NONE',  ( -70.65833882835340773, -196.5096356399514548, -360.5769090472070957 ) ) ;
#10059=CARTESIAN_POINT ( 'NONE',  ( 32.82880071992069304, -277.2140611204449101, -244.3586328017393896 ) ) ;
#10060=CARTESIAN_POINT ( 'NONE',  ( -114.3264652396838841, -272.7034455692090091, -284.0776971561411983 ) ) ;
#10061=CARTESIAN_POINT ( 'NONE',  ( 35.67938640242756776, -279.3717387606615148, -254.8156812153096666 ) ) ;
#10062=CARTESIAN_POINT ( 'NONE',  ( -109.1442272649399712, -296.0823763066272818, -256.5726169319009955 ) ) ;
#10063=CARTESIAN_POINT ( 'NONE',  ( 30.84490722477851321, -293.5199719409974932, -305.9997694829770012 ) ) ;
#10066=CARTESIAN_POINT ( 'NONE',  ( -72.98945113080966962, -296.1643055656552406, -202.7169034487176589 ) ) ;
#10067=CARTESIAN_POINT ( 'NONE',  ( -89.23794897637390022, -288.1974228851292423, -322.8322507112116568 ) ) ;
#10068=CARTESIAN_POINT ( 'NONE',  ( -42.45149074866827021, -296.9777029714415448, -344.4202532785936341 ) ) ;
#10070=CARTESIAN_POINT ( 'NONE',  ( 32.30261197297213016, -288.5576111756396926, -246.8895762823406699 ) ) ;
#10072=CARTESIAN_POINT ( 'NONE',  ( 22.01966288266718408, -293.8377689909356718, -221.6882426259114709 ) ) ;
#10073=CARTESIAN_POINT ( 'NONE',  ( -107.4157718441762626, -285.3199821643093514, -249.5067965445178686 ) ) ;
#10074=CARTESIAN_POINT ( 'NONE',  ( -84.95754812396879174, -296.2065547794595091, -210.3549538234418037 ) ) ;
#10075=CARTESIAN_POINT ( 'NONE',  ( -47.73169993441930359, -292.7262149981494872, -194.1746124373250950 ) ) ;
#10076=CARTESIAN_POINT ( 'NONE',  ( -22.21203183361346589, -292.7331521495007678, -194.8706375430522542 ) ) ;
#10077=CARTESIAN_POINT ( 'NONE',  ( -5.790510541521365795, -288.7920068999575847, -336.1906131971953187 ) ) ;
#10080=CARTESIAN_POINT ( 'NONE',  ( -112.7458507401992733, -274.5437195739473282, -264.7578475319475046 ) ) ;
#10081=CARTESIAN_POINT ( 'NONE',  ( -97.49169456466592010, -271.9848197135761438, -222.9270912740024357 ) ) ;
#10082=CARTESIAN_POINT ( 'NONE',  ( -2.326675228930831896, -281.6355269625391884, -334.6977382692795686 ) ) ;
#10084=CARTESIAN_POINT ( 'NONE',  ( -51.30760475743491611, -276.7337858303380926, -346.0214141156695291 ) ) ;
#10085=CARTESIAN_POINT ( 'NONE',  ( -103.9181012651606153, -271.3780272389824404, -238.5173866586522138 ) ) ;
#10086=CARTESIAN_POINT ( 'NONE',  ( -88.39704607707935224, -281.1883556822812125, -216.3992670618211775 ) ) ;
#10087=CARTESIAN_POINT ( 'NONE',  ( -39.21223733438745995, -275.2154597038931456, -344.5727516631195044 ) ) ;
#10088=CARTESIAN_POINT ( 'NONE',  ( -108.9760715191731464, -297.5474499343453090, -286.3500936098838565 ) ) ;
#10089=CARTESIAN_POINT ( 'NONE',  ( -106.5325994041138244, -273.8115654333241764, -246.3605366288671803 ) ) ;
#10090=CARTESIAN_POINT ( 'NONE',  ( -43.24829040909175859, -299.5790065920785992, -194.3377250612365970 ) ) ;
#10091=CARTESIAN_POINT ( 'NONE',  ( -24.41638868785404881, -272.2363182896086187, -196.0696849548029661 ) ) ;
#10092=CARTESIAN_POINT ( 'NONE',  ( 16.80810937755174805, -293.5001679676471440, -221.1779170736596427 ) ) ;
#10093=CARTESIAN_POINT ( 'NONE',  ( -7.010937760586750223, -291.0328829448560555, -203.3132263463032245 ) ) ;
#10095=CARTESIAN_POINT ( 'NONE',  ( -89.16603447433475083, -278.2507182878662206, -327.2273229961910488 ) ) ;
#10096=CARTESIAN_POINT ( 'NONE',  ( -57.91480052647060006, -298.1122424356454417, -200.2980390700794544 ) ) ;
#10098=CARTESIAN_POINT ( 'NONE',  ( -90.11020610653490337, -282.4638122541618372, -325.8303726090314285 ) ) ;
#10099=CARTESIAN_POINT ( 'NONE',  ( 21.74668994224522933, -296.1889464478860532, -316.8424118259868578 ) ) ;
#10101=CARTESIAN_POINT ( 'NONE',  ( -51.05817383886850536, -282.4289799527325613, -342.2769875619526943 ) ) ;
#10102=CARTESIAN_POINT ( 'NONE',  ( -96.61484122935095797, -281.9193463631676764, -316.5858210636096146 ) ) ;
#10103=CARTESIAN_POINT ( 'NONE',  ( 34.15471692889155264, -274.3555753317088488, -287.8393355101522957 ) ) ;
#10104=CARTESIAN_POINT ( 'NONE',  ( 33.33821948033345706, -283.8790948514794650, -295.5995821949775859 ) ) ;
#10108=CARTESIAN_POINT ( 'NONE',  ( -71.03058452618282104, -272.0148575401698849, -202.0127494104979746 ) ) ;
#10109=CARTESIAN_POINT ( 'NONE',  ( -87.95831559175432801, -279.7582887874198718, -325.9307739391316545 ) ) ;
#10111=CARTESIAN_POINT ( 'NONE',  ( -35.21376069421063448, -287.9987906217879754, -194.8181858442258090 ) ) ;
#10113=CARTESIAN_POINT ( 'NONE',  ( -97.53075140976511648, -287.9408460568409964, -315.1290064869051548 ) ) ;
#10114=CARTESIAN_POINT ( 'NONE',  ( 115.2448031289451222, -299.5541904835127980, -195.3611179825600175 ) ) ;
#10115=CARTESIAN_POINT ( 'NONE',  ( -78.18336557496067485, -294.4094986319782947, -331.4068473211712558 ) ) ;
#10116=CARTESIAN_POINT ( 'NONE',  ( -51.00161388006192453, -287.3679922815639998, -343.3812852127429096 ) ) ;
#10117=CARTESIAN_POINT ( 'NONE',  ( 163.5244876965996923, 234.8495348041943487, -191.6304063886470317 ) ) ;
#10118=CARTESIAN_POINT ( 'NONE',  ( -105.7715854310686723, -294.1480482822815929, -301.1859095118218761 ) ) ;
#10119=CARTESIAN_POINT ( 'NONE',  ( 33.22569780964552422, -285.6581705565193943, -241.1893890864233754 ) ) ;
#10120=CARTESIAN_POINT ( 'NONE',  ( 13.87579997193738457, -282.3847970942553047, -217.1560524550129401 ) ) ;
#10121=CARTESIAN_POINT ( 'NONE',  ( -97.25939844816508639, -282.1593267596914529, -317.0927287541347255 ) ) ;
#10122=CARTESIAN_POINT ( 'NONE',  ( -50.75146506802662572, -289.2281088185788462, -342.1705713351223039 ) ) ;
#10123=CARTESIAN_POINT ( 'NONE',  ( 20.12486279696889113, -282.3331824380979924, -224.3940747368134794 ) ) ;
#10124=CARTESIAN_POINT ( 'NONE',  ( 33.80958396006374045, -282.5798754056833673, -287.4466660891641254 ) ) ;
#10125=CARTESIAN_POINT ( 'NONE',  ( -3.770357505852217184, -290.5914139266557186, -337.8392912137360327 ) ) ;
#10126=CARTESIAN_POINT ( 'NONE',  ( -9.112445462621307612, -298.5631240970153044, -193.3603398670499018 ) ) ;
#10128=CARTESIAN_POINT ( 'NONE',  ( 31.85528348125702536, -275.9871838248251947, -304.2579613512853030 ) ) ;
#10129=CARTESIAN_POINT ( 'NONE',  ( 26.23587654574072658, -295.0036021948311031, -231.1511717593713229 ) ) ;
#10131=CARTESIAN_POINT ( 'NONE',  ( 10.64812456238590066, -284.9090924074130271, -330.4860931364851808 ) ) ;
#10132=CARTESIAN_POINT ( 'NONE',  ( 31.33417417030334562, -273.9515086924911316, -300.9168492442818774 ) ) ;
#10134=CARTESIAN_POINT ( 'NONE',  ( -82.48011783106134942, -295.8474271871073142, -208.9036852808880269 ) ) ;
#10135=CARTESIAN_POINT ( 'NONE',  ( -109.7193533372791023, -291.9632885458884175, -284.8449515112957897 ) ) ;
#10136=CARTESIAN_POINT ( 'NONE',  ( -21.90442576873983782, -273.6038279701614329, -198.9077539737049278 ) ) ;
#10137=CARTESIAN_POINT ( 'NONE',  ( -107.6073616987122961, -291.7785837474815480, -292.7433668894856282 ) ) ;
#10138=CARTESIAN_POINT ( 'NONE',  ( -32.15253962783823027, -293.0604326010470686, -197.2972348126272664 ) ) ;
#10139=CARTESIAN_POINT ( 'NONE',  ( -93.31092270817983092, -285.6314681143583130, -318.8099351676286801 ) ) ;
#10140=CARTESIAN_POINT ( 'NONE',  ( -88.27036707920395031, -292.7803576116512545, -213.3972946026031536 ) ) ;
#10141=CARTESIAN_POINT ( 'NONE',  ( -68.14567209144453841, -292.9712162624673510, -200.3153229453337474 ) ) ;
#10142=CARTESIAN_POINT ( 'NONE',  ( -23.52091616408201702, -294.7039990168211148, -342.0924676533860520 ) ) ;
#10143=CARTESIAN_POINT ( 'NONE',  ( 36.53301821903620805, -289.3823685584699206, -257.1255174045505782 ) ) ;
#10144=CARTESIAN_POINT ( 'NONE',  ( 30.72081916722495620, -281.2525881705676056, -234.2405979524541522 ) ) ;
#10145=CARTESIAN_POINT ( 'NONE',  ( -59.69825073501958457, -295.8447726425897599, -198.1297826147653609 ) ) ;
#10146=CARTESIAN_POINT ( 'NONE',  ( -73.61113752822717515, -285.4180740325126635, -202.3791087334140002 ) ) ;
#10147=CARTESIAN_POINT ( 'NONE',  ( -4.316170957139710218, -278.5946439040762357, -337.3167994299263910 ) ) ;
#10148=CARTESIAN_POINT ( 'NONE',  ( -67.96394637331074762, -282.2583143925389209, -337.0650049825287056 ) ) ;
#10149=CARTESIAN_POINT ( 'NONE',  ( 0.5342371799079419503, -284.5567248701766516, -205.6127680648015996 ) ) ;
#10150=CARTESIAN_POINT ( 'NONE',  ( -73.52809004499295042, -275.6665682240818001, -336.9405167085677704 ) ) ;
#10151=CARTESIAN_POINT ( 'NONE',  ( -90.79075242949535607, -283.3441026381856886, -320.1726352228607198 ) ) ;
#10152=CARTESIAN_POINT ( 'NONE',  ( -92.79695670519626560, -280.4841258988446953, -217.4390897427107916 ) ) ;
#10153=CARTESIAN_POINT ( 'NONE',  ( 39.46685440826993130, -286.6259363707403054, -271.5596149658285299 ) ) ;
#10154=CARTESIAN_POINT ( 'NONE',  ( 36.65600694997950626, -295.3532716960980906, -273.5100338923014647 ) ) ;
#10155=CARTESIAN_POINT ( 'NONE',  ( 13.41624474028927949, -276.3482778430423537, -213.4569064507844018 ) ) ;
#10156=CARTESIAN_POINT ( 'NONE',  ( 38.89054924633138910, -276.9488411776949874, -276.8374153150747929 ) ) ;
#10157=CARTESIAN_POINT ( 'NONE',  ( -107.1172517035466427, -278.0992445922971683, -291.9866930412447346 ) ) ;
#10158=CARTESIAN_POINT ( 'NONE',  ( -50.29569844190492489, -299.8865635541124561, -196.6575064599604445 ) ) ;
#10159=CARTESIAN_POINT ( 'NONE',  ( 3.467602521227912238, -284.6021483056375700, -207.6344949091392209 ) ) ;
#10160=CARTESIAN_POINT ( 'NONE',  ( -113.4512549875592669, -292.1053734450758270, -274.0727312007828687 ) ) ;
#10161=CARTESIAN_POINT ( 'NONE',  ( 22.84956097576515788, -291.8914287828226293, -228.4911966137762249 ) ) ;
#10163=CARTESIAN_POINT ( 'NONE',  ( -41.58982485106410110, -291.6640339373761890, -197.4137883815997441 ) ) ;
#10165=CARTESIAN_POINT ( 'NONE',  ( 10.04777681131517753, -289.4963247613467843, -330.7257015966046652 ) ) ;
#10166=CARTESIAN_POINT ( 'NONE',  ( -106.5439089563936363, -279.5180439181236807, -246.6483046272178399 ) ) ;
#10167=CARTESIAN_POINT ( 'NONE',  ( -95.32831459019224951, -296.1539164530156540, -220.0917893130943526 ) ) ;
#10168=CARTESIAN_POINT ( 'NONE',  ( 36.29019357390585299, -288.4827483429384642, -292.5802086880315187 ) ) ;
#10169=CARTESIAN_POINT ( 'NONE',  ( 7.528161383712674848, -286.9787604703238912, -207.7459693148948645 ) ) ;
#10170=CARTESIAN_POINT ( 'NONE',  ( -108.1126704104220408, -284.6480869448288331, -288.3488152268273552 ) ) ;
#10171=CARTESIAN_POINT ( 'NONE',  ( -63.92340429282429426, -182.6668603218660110, -362.3860721358306591 ) ) ;
#10172=CARTESIAN_POINT ( 'NONE',  ( -114.2273371156044419, -271.8154644092875287, -270.3517381826829364 ) ) ;
#10173=CARTESIAN_POINT ( 'NONE',  ( -105.9079042852521724, -259.8726411093065281, -315.4770811649867142 ) ) ;
#10174=CARTESIAN_POINT ( 'NONE',  ( 7.671714976775490413, -275.6170801770783783, -328.1005658895440433 ) ) ;
#10175=CARTESIAN_POINT ( 'NONE',  ( -96.34996190552394069, -276.8651456401346991, -313.8821771061226400 ) ) ;
#10176=CARTESIAN_POINT ( 'NONE',  ( -36.17924183282816841, -297.5739966270660943, -193.4227500555989820 ) ) ;
#10177=CARTESIAN_POINT ( 'NONE',  ( -92.70013282893863504, -239.9236592119154068, -339.3243185181465833 ) ) ;
#10179=CARTESIAN_POINT ( 'NONE',  ( -112.0068190795022360, -277.0269596698151986, -287.0469888637583722 ) ) ;
#10180=CARTESIAN_POINT ( 'NONE',  ( -56.07532559092211244, -289.7922409103848622, -341.0326937406983348 ) ) ;
#10181=CARTESIAN_POINT ( 'NONE',  ( -54.56892408893858715, -298.6390384708890906, -195.4786662692471850 ) ) ;
#10182=CARTESIAN_POINT ( 'NONE',  ( -9.144628575790221703, -298.8886658643957617, -193.4203677221946123 ) ) ;
#10183=CARTESIAN_POINT ( 'NONE',  ( -84.47648351393847577, -295.8887955996117967, -326.1707564084852038 ) ) ;
#10185=CARTESIAN_POINT ( 'NONE',  ( -67.11819910758798358, -279.3596221247182712, -339.8065952184603589 ) ) ;
#10186=CARTESIAN_POINT ( 'NONE',  ( 38.60608843914693011, -281.2148746239572574, -282.7502950367433527 ) ) ;
#10187=CARTESIAN_POINT ( 'NONE',  ( -95.50993420718145899, -279.0067352305165969, -314.9781844332607648 ) ) ;
#10188=CARTESIAN_POINT ( 'NONE',  ( -17.59929120633848498, -278.5610087195860274, -343.7383031384256924 ) ) ;
#10189=CARTESIAN_POINT ( 'NONE',  ( -103.0503548012665220, -295.5743320823794988, -237.1154376743350554 ) ) ;
#10191=CARTESIAN_POINT ( 'NONE',  ( -109.0428824163552122, -278.5371153705501683, -284.1362938232264810 ) ) ;
#10192=CARTESIAN_POINT ( 'NONE',  ( -46.87112713944789277, -274.7368936531498207, -194.1157978571005742 ) ) ;
#10193=CARTESIAN_POINT ( 'NONE',  ( -36.11167595217053616, -287.7218987114288211, -346.8711073633154456 ) ) ;
#10194=CARTESIAN_POINT ( 'NONE',  ( -80.13080328560668875, -275.4735302345370656, -208.7019593804574242 ) ) ;
#10195=CARTESIAN_POINT ( 'NONE',  ( -5.546632951704859593, -275.2167925460005904, -339.8426263003461258 ) ) ;
#10197=CARTESIAN_POINT ( 'NONE',  ( -26.46094893164605111, -288.1074540088904428, -342.7601267447482201 ) ) ;
#10198=CARTESIAN_POINT ( 'NONE',  ( -93.83920180759402285, -284.6126480565598058, -218.1165754562210282 ) ) ;
#10199=CARTESIAN_POINT ( 'NONE',  ( 26.42078663225346347, -280.3023481343462890, -308.0431775669642889 ) ) ;
#10200=CARTESIAN_POINT ( 'NONE',  ( 34.91624772855234227, -279.9436624269526988, -256.3603788803147836 ) ) ;
#10201=CARTESIAN_POINT ( 'NONE',  ( -96.90372463458312779, -283.2466710020319169, -225.7104803923780025 ) ) ;
#10202=CARTESIAN_POINT ( 'NONE',  ( 35.61719817010499867, -289.7761356342125509, -287.7933291413360166 ) ) ;
#10203=CARTESIAN_POINT ( 'NONE',  ( -51.92116565394568539, -281.0666257315007783, -198.3746223163297202 ) ) ;
#10204=CARTESIAN_POINT ( 'NONE',  ( -91.70447742415792902, -271.2771939939169670, -218.6733493027779502 ) ) ;
#10205=CARTESIAN_POINT ( 'NONE',  ( -8.362205511353741016, -281.0790322659028107, -340.8913788330370949 ) ) ;
#10206=CARTESIAN_POINT ( 'NONE',  ( 36.35513471837756327, -295.3735751972777166, -256.4407305996601281 ) ) ;
#10207=CARTESIAN_POINT ( 'NONE',  ( -61.70127681933101371, -277.9798863685323909, -198.3293505369994421 ) ) ;
#10208=CARTESIAN_POINT ( 'NONE',  ( -93.02351920001959229, -285.8494174591913293, -320.8734022832099413 ) ) ;
#10211=CARTESIAN_POINT ( 'NONE',  ( -30.84590118463275488, -294.0536633378663964, -195.0290780358346012 ) ) ;
#10212=CARTESIAN_POINT ( 'NONE',  ( -26.76394431292573728, -274.9174345958816161, -344.6114494878838173 ) ) ;
#10213=CARTESIAN_POINT ( 'NONE',  ( 38.81658475733406988, -286.6214677874908716, -260.1594287254835649 ) ) ;
#10214=CARTESIAN_POINT ( 'NONE',  ( -108.5181154060295370, -289.2069024782649080, -250.8583406240022953 ) ) ;
#10216=CARTESIAN_POINT ( 'NONE',  ( -26.96834898235329447, -275.6023107238194143, -343.1185029215001236 ) ) ;
#10217=CARTESIAN_POINT ( 'NONE',  ( 4.493271659766628900, -292.6205742437894060, -331.6856694591111250 ) ) ;
#10218=CARTESIAN_POINT ( 'NONE',  ( -109.1409294045881921, -291.6610567551922486, -286.1075840467784133 ) ) ;
#10221=CARTESIAN_POINT ( 'NONE',  ( -2.356313950823147430, -290.9863782981959730, -202.5325314325094155 ) ) ;
#10222=CARTESIAN_POINT ( 'NONE',  ( -98.02524546373331304, -286.7313162073454009, -228.3393937628766537 ) ) ;
#10223=CARTESIAN_POINT ( 'NONE',  ( -57.04997751865148814, -287.5426944628267165, -343.8018626579952866 ) ) ;
#10224=CARTESIAN_POINT ( 'NONE',  ( 34.56795388107262568, -288.7728585527140694, -254.7285692698352761 ) ) ;
#10226=CARTESIAN_POINT ( 'NONE',  ( 32.42449883106665709, -288.0631121276574618, -248.2901417484223998 ) ) ;
#10227=CARTESIAN_POINT ( 'NONE',  ( 36.18473302662236790, -295.7436520320890736, -286.9200640117798571 ) ) ;
#10229=CARTESIAN_POINT ( 'NONE',  ( 38.95335154249851684, -288.8434771316233878, -277.2221535033768305 ) ) ;
#10230=CARTESIAN_POINT ( 'NONE',  ( -28.78878386451603077, -275.0244982364519046, -345.4880653501502366 ) ) ;
#10231=CARTESIAN_POINT ( 'NONE',  ( -112.4628415868304927, -278.6751479787206449, -287.1705914307327134 ) ) ;
#10232=CARTESIAN_POINT ( 'NONE',  ( -19.75692733029804771, -279.9388520060445558, -195.3629160498394413 ) ) ;
#10233=CARTESIAN_POINT ( 'NONE',  ( -110.5503374789901443, -274.6503120203589106, -256.6012278311616797 ) ) ;
#10235=CARTESIAN_POINT ( 'NONE',  ( -78.11557340748808542, -283.5042462359920705, -207.3511836032612337 ) ) ;
#10237=CARTESIAN_POINT ( 'NONE',  ( -102.9596153327663899, -276.2267463756935513, -305.0764558297605049 ) ) ;
#10238=CARTESIAN_POINT ( 'NONE',  ( 21.80942542596930522, -280.1846917477959096, -316.4920030215609472 ) ) ;
#10240=CARTESIAN_POINT ( 'NONE',  ( -64.86324294991916872, -275.8849138629798858, -341.5876313529131494 ) ) ;
#10241=CARTESIAN_POINT ( 'NONE',  ( -109.8205513100066923, -297.8972559847620687, -283.7547328870899719 ) ) ;
#10242=CARTESIAN_POINT ( 'NONE',  ( -24.59853707242006138, -281.8136528006235153, -346.0397750232514227 ) ) ;
#10243=CARTESIAN_POINT ( 'NONE',  ( -109.5930965613321320, -297.3360860732462925, -282.3254049177900811 ) ) ;
#10244=CARTESIAN_POINT ( 'NONE',  ( -95.20915907490611119, -298.5483749017658965, -220.2354958050128459 ) ) ;
#10245=CARTESIAN_POINT ( 'NONE',  ( -38.07831613456096420, -273.7093883448439442, -197.3436893526007907 ) ) ;
#10246=CARTESIAN_POINT ( 'NONE',  ( 34.53876013362178554, -295.2744938962945298, -248.7767584772300893 ) ) ;
#10247=CARTESIAN_POINT ( 'NONE',  ( 39.57750989701042243, -287.6619923767982527, -265.8162808339412209 ) ) ;
#10249=CARTESIAN_POINT ( 'NONE',  ( -110.3335092408794793, -276.8818024192555072, -250.7789467683004148 ) ) ;
#10250=CARTESIAN_POINT ( 'NONE',  ( -103.7994992477873382, -289.8781369429692063, -309.3556701720384581 ) ) ;
#10251=CARTESIAN_POINT ( 'NONE',  ( 33.94209871645041687, -286.3893603965388479, -253.5131804390862840 ) ) ;
#10253=CARTESIAN_POINT ( 'NONE',  ( 32.60700415657181850, -291.1984148600584490, -243.1586569170810037 ) ) ;
#10255=CARTESIAN_POINT ( 'NONE',  ( -87.49538389815894845, -233.3606102865802825, -350.3678815354037965 ) ) ;
#10256=CARTESIAN_POINT ( 'NONE',  ( -53.42817283331326195, -288.7717729141947416, -341.6297214300688552 ) ) ;
#10258=CARTESIAN_POINT ( 'NONE',  ( -95.14962286871472941, -284.8081800909218373, -320.8691795352419263 ) ) ;
#10259=CARTESIAN_POINT ( 'NONE',  ( 6.372108086694794338, -291.6889415811791082, -207.2586363850788302 ) ) ;
#10260=CARTESIAN_POINT ( 'NONE',  ( 10.50148642365074458, -282.0119367044794103, -210.5912354193176270 ) ) ;
#10261=CARTESIAN_POINT ( 'NONE',  ( -29.44676271388765443, -282.7828264192551160, -342.9834478464072731 ) ) ;
#10262=CARTESIAN_POINT ( 'NONE',  ( -60.14808920178801799, -297.7646175120970042, -196.7605850772471285 ) ) ;
#10263=CARTESIAN_POINT ( 'NONE',  ( -29.95685567321685028, -275.4627549194695462, -197.2399339783096366 ) ) ;
#10264=CARTESIAN_POINT ( 'NONE',  ( 23.15217351307708071, -290.9737571614758735, -226.6090854255345732 ) ) ;
#10265=CARTESIAN_POINT ( 'NONE',  ( 31.49601424749674194, -274.0093413072679027, -244.8954629979639037 ) ) ;
#10268=CARTESIAN_POINT ( 'NONE',  ( -106.9193925465138619, -286.8187775050571986, -243.8987123139515916 ) ) ;
#10269=CARTESIAN_POINT ( 'NONE',  ( -3.353359851643989309, -295.6936313495563695, -339.1236478617678358 ) ) ;
#10270=CARTESIAN_POINT ( 'NONE',  ( -110.0967273144564729, -285.3038630400230886, -262.7476688479676454 ) ) ;
#10272=CARTESIAN_POINT ( 'NONE',  ( -42.80143333554335783, -276.1782196752573668, -346.9314224506559867 ) ) ;
#10273=CARTESIAN_POINT ( 'NONE',  ( 33.22756055264529351, -293.8137437942107795, -239.8112860147130618 ) ) ;
#10274=CARTESIAN_POINT ( 'NONE',  ( 36.89321148757449720, -285.8842855372855638, -285.5098268696603441 ) ) ;
#10275=CARTESIAN_POINT ( 'NONE',  ( -61.68591932957613011, -292.0776848538222339, -197.2768761179004002 ) ) ;
#10276=CARTESIAN_POINT ( 'NONE',  ( -105.1310912312631274, -290.5206457733049774, -297.6387637713704635 ) ) ;
#10279=CARTESIAN_POINT ( 'NONE',  ( -93.27324509058188085, -239.1325559268020413, -338.6579388652390890 ) ) ;
#10280=CARTESIAN_POINT ( 'NONE',  ( -108.6480783087754673, -285.7235663197366762, -297.6764020543627112 ) ) ;
#10281=CARTESIAN_POINT ( 'NONE',  ( -88.47809603358389552, -270.9094976428775681, -206.1857440867352693 ) ) ;
#10283=CARTESIAN_POINT ( 'NONE',  ( -76.30300386764839971, -282.5063803985242998, -332.5198139222908935 ) ) ;
#10284=CARTESIAN_POINT ( 'NONE',  ( -101.8711769383539973, -278.7713472362274274, -228.2921695624654319 ) ) ;
#10285=CARTESIAN_POINT ( 'NONE',  ( 19.91308581191904992, -284.2201907251176181, -318.5673018594951600 ) ) ;
#10286=CARTESIAN_POINT ( 'NONE',  ( -37.46467321658223426, -140.8945144798868796, -363.2317121015391876 ) ) ;
#10287=CARTESIAN_POINT ( 'NONE',  ( 15.33410500464692916, -280.8999378708354584, -325.7133161811123614 ) ) ;
#10288=CARTESIAN_POINT ( 'NONE',  ( -10.12732785420929993, -284.4292567008990886, -200.8402730129305667 ) ) ;
#10289=CARTESIAN_POINT ( 'NONE',  ( -36.92663226300399515, -299.8174149814702218, -194.3743222947530285 ) ) ;
#10290=CARTESIAN_POINT ( 'NONE',  ( -103.9901835675098170, -296.6401548799878469, -300.4174900717001151 ) ) ;
#10292=CARTESIAN_POINT ( 'NONE',  ( 36.02814424497211832, -292.1706409147439558, -265.2989475582161845 ) ) ;
#10293=CARTESIAN_POINT ( 'NONE',  ( -87.02300592960000358, -278.3740139169520944, -329.1255920172828837 ) ) ;
#10294=CARTESIAN_POINT ( 'NONE',  ( 7.330913109455482690, -274.6808826745287320, -212.6258806787310505 ) ) ;
#10295=CARTESIAN_POINT ( 'NONE',  ( 35.76380224712765710, -274.7649475973900053, -293.5360620422601414 ) ) ;
#10297=CARTESIAN_POINT ( 'NONE',  ( -86.98819434208871826, -271.3613346296446593, -214.0767188238760923 ) ) ;
#10298=ADVANCED_FACE ( 'NONE', ( #74641 ), #39770, .T. ) ;
#10299=CARTESIAN_POINT ( 'NONE',  ( -66.68128284574058284, -296.8542974108967201, -340.9287008893612665 ) ) ;
#10302=CARTESIAN_POINT ( 'NONE',  ( -108.0556988070586186, -285.3769238926561798, -289.7412608358204693 ) ) ;
#10303=CARTESIAN_POINT ( 'NONE',  ( -19.13912501052385196, -284.5813070729971059, -344.1896083012179020 ) ) ;
#10304=CARTESIAN_POINT ( 'NONE',  ( -85.78750485434918005, -284.7091102478266862, -215.5495495058500524 ) ) ;
#10305=CARTESIAN_POINT ( 'NONE',  ( 18.90505728240352212, -274.6240509143686381, -318.1391746373007550 ) ) ;
#10306=CARTESIAN_POINT ( 'NONE',  ( -0.6207420685548373784, -284.4191026330416321, -334.8780670751054913 ) ) ;
#10307=CARTESIAN_POINT ( 'NONE',  ( -111.0858159587314304, -277.0286215410363297, -270.6213641411571302 ) ) ;
#10308=CARTESIAN_POINT ( 'NONE',  ( -35.09444310858130223, -278.1029459916901487, -343.6357787480302477 ) ) ;
#10310=CARTESIAN_POINT ( 'NONE',  ( -113.0790570439091454, -279.5174289858325665, -257.3991895727211272 ) ) ;
#10311=CARTESIAN_POINT ( 'NONE',  ( 21.91929506839649022, -281.3843462366525046, -221.2931920857381556 ) ) ;
#10316=CARTESIAN_POINT ( 'NONE',  ( 34.66753030953182702, -289.1094158056665151, -246.6355643639198263 ) ) ;
#10317=CARTESIAN_POINT ( 'NONE',  ( -69.31890438994363990, -296.8174145899420751, -204.5579255435971504 ) ) ;
#10318=CARTESIAN_POINT ( 'NONE',  ( -111.8937015277938229, -290.1375104559436977, -251.4583844874519514 ) ) ;
#10319=CARTESIAN_POINT ( 'NONE',  ( 35.75654100019524861, -285.9440182258103391, -282.0443685116068195 ) ) ;
#10320=CARTESIAN_POINT ( 'NONE',  ( -30.45823730249263050, -284.7154833707213015, -197.0433212968430894 ) ) ;
#10321=CARTESIAN_POINT ( 'NONE',  ( -102.5463514248387611, -288.3197446232850893, -305.4887994554308079 ) ) ;
#10323=CARTESIAN_POINT ( 'NONE',  ( 9.270903025119748619, -287.9144461534589823, -213.6654767840914531 ) ) ;
#10324=CARTESIAN_POINT ( 'NONE',  ( -42.68965519938510766, -275.1194821093689029, -345.1702085131020112 ) ) ;
#10325=CARTESIAN_POINT ( 'NONE',  ( 26.76066079865502090, -286.4993076210790832, -311.6570068035015879 ) ) ;
#10326=CARTESIAN_POINT ( 'NONE',  ( -0.7157412622314297534, -288.5387744371663530, -204.8977065826459238 ) ) ;
#10327=CARTESIAN_POINT ( 'NONE',  ( 33.33962356623377588, -285.8846397867724818, -296.0893293781351190 ) ) ;
#10328=CARTESIAN_POINT ( 'NONE',  ( -29.40728608658041665, -283.8905798774223967, -343.2159982785695433 ) ) ;
#10329=CARTESIAN_POINT ( 'NONE',  ( -62.13433141903735901, -291.3738143722598579, -341.3763799180966885 ) ) ;
#10332=CARTESIAN_POINT ( 'NONE',  ( -48.77666737481985137, -299.8279071822468609, -195.6187238604632626 ) ) ;
#10333=CARTESIAN_POINT ( 'NONE',  ( 11.18383693049203309, -280.3803540264718208, -327.6156944722021649 ) ) ;
#10334=CARTESIAN_POINT ( 'NONE',  ( -36.37011880712959311, -291.2612149078244670, -193.5157311925835870 ) ) ;
#10335=CARTESIAN_POINT ( 'NONE',  ( -107.4605578002511805, -295.2561064065175742, -247.1821617651352483 ) ) ;
#10336=CARTESIAN_POINT ( 'NONE',  ( 31.81298249496248332, -280.5678454737161474, -295.3886556471273366 ) ) ;
#10337=CARTESIAN_POINT ( 'NONE',  ( 31.51597371762045086, -273.2586846197522163, -241.9425349285816651 ) ) ;
#10338=CARTESIAN_POINT ( 'NONE',  ( -90.75420235055038631, -297.1443569384984471, -320.9155540161502813 ) ) ;
#10340=CARTESIAN_POINT ( 'NONE',  ( -31.95084658018009094, -296.5983711020932105, -194.0558108093565295 ) ) ;
#10341=CARTESIAN_POINT ( 'NONE',  ( 37.07360994593462777, -291.9868439027692943, -285.7343298523142607 ) ) ;
#10342=CARTESIAN_POINT ( 'NONE',  ( -72.92767687482512429, -292.9965010862782151, -205.8910156031611791 ) ) ;
#10344=CARTESIAN_POINT ( 'NONE',  ( 34.87167903853408291, -294.1994283913480217, -258.5427603614354553 ) ) ;
#10346=CARTESIAN_POINT ( 'NONE',  ( -33.17544088809017211, -281.0200632758420625, -345.6139159875704081 ) ) ;
#10347=CARTESIAN_POINT ( 'NONE',  ( 32.34680181013401068, -293.8402056837952614, -292.0984751725993647 ) ) ;
#10348=CARTESIAN_POINT ( 'NONE',  ( 37.19180675334335007, -281.7941203473868654, -289.6938971918879133 ) ) ;
#10349=CARTESIAN_POINT ( 'NONE',  ( -14.68332004295251991, -282.2635479267149776, -198.2235943804611225 ) ) ;
#10350=CARTESIAN_POINT ( 'NONE',  ( -23.78545685063492954, -285.8874039504225948, -194.5311109862090007 ) ) ;
#10351=CARTESIAN_POINT ( 'NONE',  ( -112.1399717792138375, -288.5055117233392252, -273.9726583450377007 ) ) ;
#10353=CARTESIAN_POINT ( 'NONE',  ( -5.760299601673096959, -281.1242569195130159, -339.8256621444779171 ) ) ;
#10354=CARTESIAN_POINT ( 'NONE',  ( 19.38629957467626852, -287.1769087218513050, -321.9890706773002762 ) ) ;
#10356=CARTESIAN_POINT ( 'NONE',  ( -23.34738004351993013, -296.4705231276534505, -342.8743100118807661 ) ) ;
#10357=CARTESIAN_POINT ( 'NONE',  ( 36.67255589461953491, -277.2168581614968161, -289.3478554576635133 ) ) ;
#10358=CARTESIAN_POINT ( 'NONE',  ( 37.18600708022069767, -291.7145815150284989, -281.4978886730869476 ) ) ;
#10359=CARTESIAN_POINT ( 'NONE',  ( -95.62606371277487938, -278.8368537839979240, -226.3514971737146482 ) ) ;
#10360=CARTESIAN_POINT ( 'NONE',  ( -8.513188748562830810, -292.5859176008610802, -198.9614195507538454 ) ) ;
#10361=CARTESIAN_POINT ( 'NONE',  ( -112.8858941111470813, -282.6729117403816645, -267.1507352859035791 ) ) ;
#10362=CARTESIAN_POINT ( 'NONE',  ( -34.34483341811321822, -279.0146256576710471, -345.3012236743965673 ) ) ;
#10363=CARTESIAN_POINT ( 'NONE',  ( 19.00648301982591093, -293.2722682122375204, -317.1402875428370862 ) ) ;
#10364=CARTESIAN_POINT ( 'NONE',  ( -32.05918893263172720, -296.1181216209474769, -195.3629102556025998 ) ) ;
#10367=CARTESIAN_POINT ( 'NONE',  ( -104.8683284471737664, -280.9538156128166975, -238.4275723611758337 ) ) ;
#10368=CARTESIAN_POINT ( 'NONE',  ( 33.70908018399811112, -292.8347742835921963, -253.2848703240079260 ) ) ;
#10370=CARTESIAN_POINT ( 'NONE',  ( -67.68488546085839630, -289.1237833571631768, -207.2794874003663779 ) ) ;
#10371=CARTESIAN_POINT ( 'NONE',  ( -40.41878504565425345, -297.0732436160367911, -193.6061401274947684 ) ) ;
#10372=CARTESIAN_POINT ( 'NONE',  ( -29.53004843166437610, -287.4643031591140243, -194.2541119313540037 ) ) ;
#10373=CARTESIAN_POINT ( 'NONE',  ( -34.58012825362258269, -288.8499472898386102, -343.3584463376331541 ) ) ;
#10374=CARTESIAN_POINT ( 'NONE',  ( -91.82231812343631816, -280.7771267792291496, -220.7368294145919947 ) ) ;
#10375=CARTESIAN_POINT ( 'NONE',  ( -107.0688381692570488, -274.4703356156919085, -246.1833051132217918 ) ) ;
#10376=CARTESIAN_POINT ( 'NONE',  ( -93.38350063318468131, -278.0172278784405648, -222.9450911111168239 ) ) ;
#10378=CARTESIAN_POINT ( 'NONE',  ( -34.04382328403392677, -297.7591056291649920, -193.3824422723413079 ) ) ;
#10379=CARTESIAN_POINT ( 'NONE',  ( -75.74301641984335731, -293.4558982481039493, -206.5306123059871481 ) ) ;
#10380=CARTESIAN_POINT ( 'NONE',  ( 38.02829655723240165, -295.2940243517769545, -281.5773568860684577 ) ) ;
#10382=CARTESIAN_POINT ( 'NONE',  ( -107.4954547383039909, -291.4756055206681822, -249.7656581408620013 ) ) ;
#10386=CARTESIAN_POINT ( 'NONE',  ( 36.22830416734981185, -291.4615720379416643, -252.2569761382982279 ) ) ;
#10388=CARTESIAN_POINT ( 'NONE',  ( -33.80656489309921398, -297.7643252171774293, -197.3401806514473549 ) ) ;
#10391=CARTESIAN_POINT ( 'NONE',  ( -97.81081234157554150, -292.6991598215076920, -223.7975759294687919 ) ) ;
#10392=CARTESIAN_POINT ( 'NONE',  ( -119.3990491898856732, -293.0519495502701943, -270.3937649182068412 ) ) ;
#10393=CARTESIAN_POINT ( 'NONE',  ( -16.68977181470062732, -288.3195797923462464, -198.3797194067700502 ) ) ;
#10394=CARTESIAN_POINT ( 'NONE',  ( -4.480570436723880334, -272.4859908324981461, -203.1147001390953903 ) ) ;
#10395=CARTESIAN_POINT ( 'NONE',  ( 20.09463257291801597, -276.8141380411534556, -223.0073231278088315 ) ) ;
#10396=CARTESIAN_POINT ( 'NONE',  ( -17.01637942941059478, -290.3963254354550259, -198.6960619842710969 ) ) ;
#10397=CARTESIAN_POINT ( 'NONE',  ( -11.94606309947037204, -282.2395003475567705, -198.9242012499309453 ) ) ;
#10399=CARTESIAN_POINT ( 'NONE',  ( -38.89555298335665867, -282.4207048524811512, -343.4590434138172554 ) ) ;
#10400=CARTESIAN_POINT ( 'NONE',  ( -112.1797373119256775, -279.4214173614275296, -287.1170334106876680 ) ) ;
#10401=CARTESIAN_POINT ( 'NONE',  ( -25.44206217947374071, -278.9955218419108860, -194.6880888746761116 ) ) ;
#10402=CARTESIAN_POINT ( 'NONE',  ( 4.396380910141553855, -58.38232387978199256, -351.6302086872513541 ) ) ;
#10403=CARTESIAN_POINT ( 'NONE',  ( 36.66199927469088493, -276.7503278752630536, -290.8129213564855036 ) ) ;
#10406=CARTESIAN_POINT ( 'NONE',  ( -87.59445373597829132, -274.8859665885781283, -212.8681338081721321 ) ) ;
#10407=CARTESIAN_POINT ( 'NONE',  ( -53.28691492658256834, -279.7662352645559736, -340.3683826091709079 ) ) ;
#10411=CARTESIAN_POINT ( 'NONE',  ( -94.33596509774943684, -290.9823965034725006, -316.4683824346556662 ) ) ;
#10412=CARTESIAN_POINT ( 'NONE',  ( -108.9035566690691326, -291.9836875177282991, -296.0683934744686212 ) ) ;
#10413=CARTESIAN_POINT ( 'NONE',  ( -98.93210732212988034, -289.3568454957165272, -309.7376898216074892 ) ) ;
#10414=CARTESIAN_POINT ( 'NONE',  ( -7.361317943236533878, -285.9424251958917580, -199.4475819698151327 ) ) ;
#10416=CARTESIAN_POINT ( 'NONE',  ( 21.63709376544842655, -280.5684566432405518, -314.7434893531541888 ) ) ;
#10417=CARTESIAN_POINT ( 'NONE',  ( 16.92991528933320566, -290.1295590083218485, -321.0867030176503931 ) ) ;
#10418=CARTESIAN_POINT ( 'NONE',  ( -40.28121171501673814, -281.5696464504039227, -343.9958042750290019 ) ) ;
#10419=CARTESIAN_POINT ( 'NONE',  ( 33.20329212461374624, -282.5965481485999931, -249.7541398761201208 ) ) ;
#10420=CARTESIAN_POINT ( 'NONE',  ( 20.40384084099146733, -289.1799449687768515, -320.9602950550949458 ) ) ;
#10421=CARTESIAN_POINT ( 'NONE',  ( -81.32992359588129716, -279.9282673989548584, -211.9621379610919121 ) ) ;
#10422=CARTESIAN_POINT ( 'NONE',  ( -84.01221970299478414, -290.2221554334811913, -209.5499630389306844 ) ) ;
#10423=CARTESIAN_POINT ( 'NONE',  ( -99.22029928472194626, -285.9624415080560311, -224.7192184990594512 ) ) ;
#10424=CARTESIAN_POINT ( 'NONE',  ( -76.08116222059351230, -286.0417780232569953, -203.8258521546716793 ) ) ;
#10425=CARTESIAN_POINT ( 'NONE',  ( -107.3913212994303592, -284.4465008875876038, -290.9496140503081278 ) ) ;
#10428=CARTESIAN_POINT ( 'NONE',  ( -44.79942596471324379, -293.8192604128157654, -194.9121756299024923 ) ) ;
#10429=CARTESIAN_POINT ( 'NONE',  ( 34.00902022171862882, -291.8832910336687974, -242.6035284343190028 ) ) ;
#10430=CARTESIAN_POINT ( 'NONE',  ( 24.17553975138443434, -275.1603718483514740, -310.1917077507918634 ) ) ;
#10431=CARTESIAN_POINT ( 'NONE',  ( -79.42811998457050038, -294.9531504068605159, -334.7198473830778198 ) ) ;
#10432=CARTESIAN_POINT ( 'NONE',  ( -106.3531781858590932, -289.3753385092677490, -244.3683360026673768 ) ) ;
#10433=CARTESIAN_POINT ( 'NONE',  ( 15.01751454587202872, -292.5414745646988308, -322.7445946047343455 ) ) ;
#10434=CARTESIAN_POINT ( 'NONE',  ( -5.885295437337413560, -293.6802368486648334, -204.0326708483576965 ) ) ;
#10435=DIRECTION ( 'NONE',  ( -1.000000000000000000, -0.000000000000000000, -0.000000000000000000 ) ) ;
#10436=CARTESIAN_POINT ( 'NONE',  ( 22.53075550974246255, -290.9314232919520009, -224.8941643023447625 ) ) ;
#10437=CARTESIAN_POINT ( 'NONE',  ( 25.11433188523751170, -296.1135720362655093, -311.9081734441294884 ) ) ;
#10438=CARTESIAN_POINT ( 'NONE',  ( -26.42802519558905061, -289.8512577627943188, -342.8298730236060692 ) ) ;
#10439=CARTESIAN_POINT ( 'NONE',  ( -7.208754686653007226, -278.6387780073622480, -339.4432442664805194 ) ) ;
#10440=CARTESIAN_POINT ( 'NONE',  ( -101.7713765416022227, -276.7995399529935412, -311.8925316507010166 ) ) ;
#10441=CARTESIAN_POINT ( 'NONE',  ( -64.85585218110912820, -273.0506747801122742, -198.5396803778954506 ) ) ;
#10442=CARTESIAN_POINT ( 'NONE',  ( 27.72922961401178910, -279.1472748416293825, -234.2074418495037946 ) ) ;
#10443=CARTESIAN_POINT ( 'NONE',  ( -56.74025005335258953, -275.6979373405119418, -344.1050640318513274 ) ) ;
#10444=CARTESIAN_POINT ( 'NONE',  ( -97.59723696607882459, -294.6542228942302017, -312.4385912776602936 ) ) ;
#10445=CARTESIAN_POINT ( 'NONE',  ( -91.97293552038924247, -275.2725483744221719, -218.9574111575386439 ) ) ;
#10446=CARTESIAN_POINT ( 'NONE',  ( -39.18261759023302204, -298.8313321062738623, -197.2103693235461321 ) ) ;
#10449=CARTESIAN_POINT ( 'NONE',  ( -45.86531372870712886, -287.1796816661181992, -345.2846993941365099 ) ) ;
#10450=CARTESIAN_POINT ( 'NONE',  ( 5.178469112389147533, -274.4783030319850923, -210.9603282420799815 ) ) ;
#10451=CARTESIAN_POINT ( 'NONE',  ( 39.60432534630992052, -287.6029507991769378, -274.4229353302731056 ) ) ;
#10452=CARTESIAN_POINT ( 'NONE',  ( -86.84850476573345190, -275.3659278544479321, -213.7312673841425976 ) ) ;
#10453=CARTESIAN_POINT ( 'NONE',  ( -110.0870769161513181, -294.3254077254051140, -287.9691065984814600 ) ) ;
#10454=CARTESIAN_POINT ( 'NONE',  ( -2.974255308287749422, -281.8068451363273539, -339.1000989682818840 ) ) ;
#10456=CARTESIAN_POINT ( 'NONE',  ( -74.48243906413325988, -277.5583867571803012, -205.1443982511464981 ) ) ;
#10458=CARTESIAN_POINT ( 'NONE',  ( -66.70893448764876155, -290.4535263652925892, -203.0952570144076788 ) ) ;
#10461=CARTESIAN_POINT ( 'NONE',  ( -50.00193338202542748, -289.8905829064393629, -196.3846497186790430 ) ) ;
#10462=CARTESIAN_POINT ( 'NONE',  ( -5.021282101477411608, -276.0057029830579154, -204.1195395975817064 ) ) ;
#10463=CARTESIAN_POINT ( 'NONE',  ( 30.56188935648144422, -283.4325423727615885, -305.3997941339107456 ) ) ;
#10464=CARTESIAN_POINT ( 'NONE',  ( -94.91431266262259214, -271.3044901512987508, -221.4054459890624855 ) ) ;
#10465=CARTESIAN_POINT ( 'NONE',  ( -34.84654087315310278, -283.0199734239710097, -343.3308994947895485 ) ) ;
#10466=CARTESIAN_POINT ( 'NONE',  ( 3.239869799699233610, -276.0341177301520474, -208.9120267283728651 ) ) ;
#10467=CARTESIAN_POINT ( 'NONE',  ( 0.6876917415886037999, -275.3762750066214835, -207.8601813420770839 ) ) ;
#10469=CARTESIAN_POINT ( 'NONE',  ( -75.71220310470822312, -285.5639878299744510, -334.8628066158308911 ) ) ;
#10471=CARTESIAN_POINT ( 'NONE',  ( 204.9739665765744974, 293.8334707905521554, -54.00000000001804068 ) ) ;
#10472=CARTESIAN_POINT ( 'NONE',  ( -5.799642124202470939, -294.4820825094672045, -340.6042570169652777 ) ) ;
#10473=CARTESIAN_POINT ( 'NONE',  ( -57.87040969928217038, -287.7657409284143455, -198.5408942880984853 ) ) ;
#10475=CARTESIAN_POINT ( 'NONE',  ( -55.56934967048407970, -283.3380690714490697, -190.3538533559490702 ) ) ;
#10476=CARTESIAN_POINT ( 'NONE',  ( -59.62796332002544375, -276.5308358882868447, -343.8966963989101941 ) ) ;
#10477=CARTESIAN_POINT ( 'NONE',  ( -70.53067184166060599, -290.0217210693647303, -201.7686069082039637 ) ) ;
#10478=CARTESIAN_POINT ( 'NONE',  ( -69.09102002166399359, -287.1469252974607684, -203.8438989350652548 ) ) ;
#10479=CARTESIAN_POINT ( 'NONE',  ( -40.52725266688558037, -278.8528665413316503, -344.3185070341197047 ) ) ;
#10480=CARTESIAN_POINT ( 'NONE',  ( -89.49741724719342528, -286.7600217122122217, -214.4466133842082627 ) ) ;
#10481=CARTESIAN_POINT ( 'NONE',  ( -5.152059720449447155, -284.6287268084413427, -338.1161333162526716 ) ) ;
#10482=CARTESIAN_POINT ( 'NONE',  ( -17.35585397138957475, -276.9678040294485868, -344.7221693326229683 ) ) ;
#10483=CARTESIAN_POINT ( 'NONE',  ( -39.96507856654450563, -276.9175473676718866, -347.3294821416055242 ) ) ;
#10484=CARTESIAN_POINT ( 'NONE',  ( -111.4869238625137342, -298.5651493233611404, -263.1846805494872683 ) ) ;
#10487=CARTESIAN_POINT ( 'NONE',  ( -107.1377320441797423, -271.1813315516205876, -240.1867042516654465 ) ) ;
#10489=CARTESIAN_POINT ( 'NONE',  ( -71.68865467144316028, -277.0265573997915567, -334.8599193487440857 ) ) ;
#10490=CARTESIAN_POINT ( 'NONE',  ( 6.992617980718112136, -275.8456764013615725, -207.8262216018322874 ) ) ;
#10491=CARTESIAN_POINT ( 'NONE',  ( 23.20990409826498535, -281.2434288437601140, -317.5662879070295048 ) ) ;
#10492=CARTESIAN_POINT ( 'NONE',  ( -10.40172968695477351, -288.1686865617420494, -201.4111167750988329 ) ) ;
#10493=CARTESIAN_POINT ( 'NONE',  ( -50.33028691975509616, -296.7350564382581979, -345.6076892880706737 ) ) ;
#10494=CARTESIAN_POINT ( 'NONE',  ( -112.8099822336917981, -297.5883278254459015, -283.7962421834400288 ) ) ;
#10495=CARTESIAN_POINT ( 'NONE',  ( -0.3725905512409277698, -294.5449658588265720, -205.2823641809736159 ) ) ;
#10496=CARTESIAN_POINT ( 'NONE',  ( -11.07639805348886242, -278.3949851672785485, -200.2337590440926931 ) ) ;
#10497=CARTESIAN_POINT ( 'NONE',  ( 35.15739103849399783, -283.2538329804272053, -253.4733714793716501 ) ) ;
#10498=CARTESIAN_POINT ( 'NONE',  ( -66.10702130942968324, -295.7525589130432877, -201.7034855097575416 ) ) ;
#10499=CARTESIAN_POINT ( 'NONE',  ( -87.77662108766821802, -285.3428265017375338, -327.5521216856410547 ) ) ;
#10500=CARTESIAN_POINT ( 'NONE',  ( 35.30436796394098309, -286.3383739074523646, -260.1524026511864918 ) ) ;
#10501=CARTESIAN_POINT ( 'NONE',  ( 25.01975656489566191, -281.4983696210121025, -315.3763720174604259 ) ) ;
#10502=CARTESIAN_POINT ( 'NONE',  ( -46.52282107818741252, -155.8297569508557103, -364.8203920681885393 ) ) ;
#10504=CARTESIAN_POINT ( 'NONE',  ( 9.047192352787497782, -286.3763368047199265, -213.9682271090025552 ) ) ;
#10505=VERTEX_POINT ( 'NONE', #52387 ) ;
#10506=CARTESIAN_POINT ( 'NONE',  ( -105.5030844990899084, -285.1756352417384051, -305.6268853121133020 ) ) ;
#10507=CARTESIAN_POINT ( 'NONE',  ( 29.10352467592040426, -275.4757806086246319, -239.9548332820023404 ) ) ;
#10508=CARTESIAN_POINT ( 'NONE',  ( 18.07490898210431851, -285.6194753566368263, -217.3978533250726741 ) ) ;
#10509=CARTESIAN_POINT ( 'NONE',  ( -88.43328048440179145, -290.2758172184852015, -213.1672116141976119 ) ) ;
#10510=CARTESIAN_POINT ( 'NONE',  ( 8.396702525093648006, -281.6021369168646515, -208.6442681985528793 ) ) ;
#10512=CARTESIAN_POINT ( 'NONE',  ( -70.94685247331746325, -281.1368924751873237, -201.8527134510522103 ) ) ;
#10513=CARTESIAN_POINT ( 'NONE',  ( 36.96348791680276946, -281.6329323207564244, -250.1993700939111989 ) ) ;
#10515=CARTESIAN_POINT ( 'NONE',  ( -21.33282851196157992, -289.7666405000204009, -200.3683826091710216 ) ) ;
#10516=CARTESIAN_POINT ( 'NONE',  ( -70.42391949612618873, -196.6322980649380554, -360.5434824908751921 ) ) ;
#10518=CARTESIAN_POINT ( 'NONE',  ( -21.23418448624794408, -278.8453654274079554, -343.4936675195637577 ) ) ;
#10519=CARTESIAN_POINT ( 'NONE',  ( -64.41477511282899115, -182.3306986604505369, -361.9618145500567152 ) ) ;
#10522=CARTESIAN_POINT ( 'NONE',  ( 27.90858972870336885, -279.0875463347991854, -234.1085805025546733 ) ) ;
#10523=CARTESIAN_POINT ( 'NONE',  ( -105.8985381827449430, -296.2403504500983331, -244.8409028658976183 ) ) ;
#10524=CARTESIAN_POINT ( 'NONE',  ( -69.59164127088642715, -291.1465974760457698, -200.4935980539915477 ) ) ;
#10526=CARTESIAN_POINT ( 'NONE',  ( -36.88287069353361147, -296.6325250765249280, -193.9504510854497425 ) ) ;
#10527=CARTESIAN_POINT ( 'NONE',  ( 18.39360481804174796, -285.2699266819970489, -221.9874040553980308 ) ) ;
#10528=CARTESIAN_POINT ( 'NONE',  ( 33.80620824946854697, -295.1347719039209778, -248.9983186340460293 ) ) ;
#10529=CARTESIAN_POINT ( 'NONE',  ( 25.36281638439481867, -288.3427149551805542, -232.0285328057815946 ) ) ;
#10531=CARTESIAN_POINT ( 'NONE',  ( 37.82904797230479943, -294.2973698966376901, -254.7346436236097134 ) ) ;
#10532=CARTESIAN_POINT ( 'NONE',  ( -91.70664553050789891, -284.3463132952726937, -319.1901979379171621 ) ) ;
#10533=CARTESIAN_POINT ( 'NONE',  ( -73.08163471227459240, -296.3844663975170874, -202.5481309824065193 ) ) ;
#10534=CARTESIAN_POINT ( 'NONE',  ( -34.97564950310230358, -292.8839554507575826, -193.5459080265265470 ) ) ;
#10536=CARTESIAN_POINT ( 'NONE',  ( -19.40720996155652500, -292.7690958600406361, -195.4873527249994822 ) ) ;
#10537=CARTESIAN_POINT ( 'NONE',  ( 1.313381584854082629, -288.6866308616935726, -332.2867561485459760 ) ) ;
#10540=CARTESIAN_POINT ( 'NONE',  ( -82.25767650301071399, -299.3074145657657255, -209.2806694197529112 ) ) ;
#10541=CARTESIAN_POINT ( 'NONE',  ( -29.86230698156242269, -272.9397709358210591, -194.1242017514943541 ) ) ;
#10543=CARTESIAN_POINT ( 'NONE',  ( 33.54825666909618320, -280.8534280356370232, -288.7964247969299549 ) ) ;
#10546=CARTESIAN_POINT ( 'NONE',  ( -68.99579130527776272, -276.9650046599041389, -340.5007241235339848 ) ) ;
#10547=CARTESIAN_POINT ( 'NONE',  ( 9.501111249989374841, -297.1288287902126513, -196.6801671452016649 ) ) ;
#10548=CARTESIAN_POINT ( 'NONE',  ( -59.54220080878624799, -279.2031490689377051, -341.1989839014649419 ) ) ;
#10549=CARTESIAN_POINT ( 'NONE',  ( 22.49055342951936964, -273.0863415453952712, -226.4183493338155984 ) ) ;
#10550=CARTESIAN_POINT ( 'NONE',  ( -71.86526864358874889, -298.7902021470626437, -205.5760632716375085 ) ) ;
#10551=CARTESIAN_POINT ( 'NONE',  ( -77.69354637296220289, -298.5763254413215009, -209.0959065072013630 ) ) ;
#10552=CARTESIAN_POINT ( 'NONE',  ( -86.95697786558335451, -298.9754459570530116, -212.4576034322300586 ) ) ;
#10553=CARTESIAN_POINT ( 'NONE',  ( -75.57595720050751709, -271.5652619612874901, -205.3658806995060786 ) ) ;
#10554=CARTESIAN_POINT ( 'NONE',  ( 35.52670306924603949, -294.2804817817951175, -276.1996523395038139 ) ) ;
#10555=CARTESIAN_POINT ( 'NONE',  ( -30.73615284537430270, -290.7120126532718700, -197.0689515375237875 ) ) ;
#10557=CARTESIAN_POINT ( 'NONE',  ( -1.335848643648253953, -275.0090871333285918, -202.3676950486506030 ) ) ;
#10558=CARTESIAN_POINT ( 'NONE',  ( 94.45372940089858105, -300.0800948388032907, -197.3323955020603364 ) ) ;
#10559=CARTESIAN_POINT ( 'NONE',  ( -0.6269036817332512834, -281.2596968438467684, -337.4976553236531345 ) ) ;
#10562=CARTESIAN_POINT ( 'NONE',  ( -66.63359273667273897, -282.6430907314793899, -337.4163993105046870 ) ) ;
#10563=CARTESIAN_POINT ( 'NONE',  ( -33.18618578371622618, -280.9997982578522056, -345.4256567544264271 ) ) ;
#10564=CARTESIAN_POINT ( 'NONE',  ( -6.042364950175674210, -275.2072546392021195, -336.9762458937328802 ) ) ;
#10565=CARTESIAN_POINT ( 'NONE',  ( -4.171684523773215858, -282.4895854993828834, -203.0808589391315309 ) ) ;
#10568=CARTESIAN_POINT ( 'NONE',  ( -102.0290388320079131, -271.4844634417097495, -230.0871980611412084 ) ) ;
#10569=CARTESIAN_POINT ( 'NONE',  ( -108.0043536723064506, -280.2189563623049366, -296.1416942028620269 ) ) ;
#10572=CARTESIAN_POINT ( 'NONE',  ( -75.99974213772705411, -285.4839943146464520, -335.3438004477348500 ) ) ;
#10575=CARTESIAN_POINT ( 'NONE',  ( -64.29831819532192583, -289.7003837382890765, -200.3188087569270976 ) ) ;
#10576=CARTESIAN_POINT ( 'NONE',  ( 82.13570310075333225, -300.5876282232119365, -197.0894904801451730 ) ) ;
#10577=CARTESIAN_POINT ( 'NONE',  ( -105.1230614484717307, -295.7226269191929191, -242.2041017807349874 ) ) ;
#10578=CARTESIAN_POINT ( 'NONE',  ( -101.3813065082240712, -288.1835819321852910, -308.0096444239943594 ) ) ;
#10579=CARTESIAN_POINT ( 'NONE',  ( -117.0947446405890418, -269.4376451100752661, -283.8482964293340274 ) ) ;
#10580=CARTESIAN_POINT ( 'NONE',  ( -80.86862163996777042, -295.4611348651387175, -209.2840539585544661 ) ) ;
#10581=CARTESIAN_POINT ( 'NONE',  ( 32.08928784296128356, -285.6222640009506790, -238.5787440806087432 ) ) ;
#10582=CARTESIAN_POINT ( 'NONE',  ( 30.75188450773570281, -282.7747022875940388, -241.9058171619225845 ) ) ;
#10583=CARTESIAN_POINT ( 'NONE',  ( -2.123957662188769024, -280.8322464549225401, -337.6937596318705914 ) ) ;
#10584=CARTESIAN_POINT ( 'NONE',  ( -53.40852788821273833, -289.2640408804089702, -341.5710684510602846 ) ) ;
#10585=CARTESIAN_POINT ( 'NONE',  ( 35.14438090138292381, -282.8113116095946111, -257.6669076879501858 ) ) ;
#10586=CARTESIAN_POINT ( 'NONE',  ( 35.19149507609770922, -282.2241032295702894, -260.4173409782697490 ) ) ;
#10587=CARTESIAN_POINT ( 'NONE',  ( 21.68736377104704260, -288.8912987164727610, -223.5006587009104919 ) ) ;
#10589=CARTESIAN_POINT ( 'NONE',  ( -36.89899258508963698, -298.2242305952832453, -193.3611058027246372 ) ) ;
#10591=CARTESIAN_POINT ( 'NONE',  ( -10.34761437073554013, -274.3947278289446672, -198.1911549144437856 ) ) ;
#10592=AXIS2_PLACEMENT_3D ( 'NONE', #87106, #35997, #64458 ) ;
#10593=CARTESIAN_POINT ( 'NONE',  ( 21.46342811626096392, -294.8979961258236244, -224.3643124161924334 ) ) ;
#10595=CARTESIAN_POINT ( 'NONE',  ( -37.30987171927208124, -279.5519495502701943, -345.3611179825600175 ) ) ;
#10598=CARTESIAN_POINT ( 'NONE',  ( 35.80183551150867061, -273.7745680256415426, -287.7384755368569245 ) ) ;
#10601=CARTESIAN_POINT ( 'NONE',  ( -91.05699994692098187, -295.7042963624351160, -216.3138518182221333 ) ) ;
#10602=CARTESIAN_POINT ( 'NONE',  ( -65.84525176567159122, -273.0177052169784702, -203.0451450457143210 ) ) ;
#10603=CARTESIAN_POINT ( 'NONE',  ( -72.97905615242036959, -293.0913354385656930, -205.8003836415110470 ) ) ;
#10604=CARTESIAN_POINT ( 'NONE',  ( -88.10228824416095961, -292.2620763513778002, -217.5011454341837123 ) ) ;
#10605=CARTESIAN_POINT ( 'NONE',  ( -32.05120441753491178, -284.7446404507693956, -344.1851294501523739 ) ) ;
#10606=CARTESIAN_POINT ( 'NONE',  ( -108.9282397320278193, -292.3196627312282203, -243.4899506931130873 ) ) ;
#10607=CARTESIAN_POINT ( 'NONE',  ( -74.45443149787806192, -292.8842833087218764, -203.4586259248638100 ) ) ;
#10608=CARTESIAN_POINT ( 'NONE',  ( 32.34616958529813502, -293.6735525414015342, -292.1005020428078751 ) ) ;
#10609=CARTESIAN_POINT ( 'NONE',  ( 36.94479668947634821, -289.6860340955115589, -280.7755589985422944 ) ) ;
#10610=CARTESIAN_POINT ( 'NONE',  ( 29.28552040893277919, -281.2168826662700098, -231.7630158530184872 ) ) ;
#10611=CARTESIAN_POINT ( 'NONE',  ( -89.73160184683830209, -293.8636497118489501, -324.8814314600364241 ) ) ;
#10612=CARTESIAN_POINT ( 'NONE',  ( -16.14387518094875418, -282.6188849751607677, -344.4410763332583656 ) ) ;
#10613=CARTESIAN_POINT ( 'NONE',  ( 12.87240676034157083, -278.3275301578902372, -325.6616163387516849 ) ) ;
#10614=CARTESIAN_POINT ( 'NONE',  ( -101.0710525930141728, -276.1443054044719361, -311.4309735074156151 ) ) ;
#10616=CARTESIAN_POINT ( 'NONE',  ( -71.44315577849425836, -283.0230739108393436, -334.9759704882437745 ) ) ;
#10617=CARTESIAN_POINT ( 'NONE',  ( -9.022245195677088603, -281.6194890971141263, -199.1851586208185267 ) ) ;
#10618=CARTESIAN_POINT ( 'NONE',  ( 5.059727645143717645, -285.6686197322854355, -206.3060877940217495 ) ) ;
#10619=CARTESIAN_POINT ( 'NONE',  ( 15.58467417205010186, -294.5732435225760355, -218.5501970754897911 ) ) ;
#10620=CARTESIAN_POINT ( 'NONE',  ( 38.34547702410463188, -277.2694172178909184, -279.6301473563684112 ) ) ;
#10621=CARTESIAN_POINT ( 'NONE',  ( -7.895966841277534343, -275.7450120130596929, -199.6915263846346704 ) ) ;
#10622=CARTESIAN_POINT ( 'NONE',  ( -93.60738808868578076, -277.7259347629495778, -316.8906209122224027 ) ) ;
#10623=CARTESIAN_POINT ( 'NONE',  ( -71.32223896733360391, -299.6026364329388798, -203.6733865007713575 ) ) ;
#10624=CARTESIAN_POINT ( 'NONE',  ( 32.69931597076778473, -285.2072911839994163, -243.8654259879708661 ) ) ;
#10625=CARTESIAN_POINT ( 'NONE',  ( -61.58893174056260023, -295.0253479603252913, -343.4772017382548484 ) ) ;
#10626=CARTESIAN_POINT ( 'NONE',  ( -111.1420792891184988, -291.9117578233698964, -289.3854632699785725 ) ) ;
#10627=CARTESIAN_POINT ( 'NONE',  ( 9.055060521613025770, -291.6264290658095319, -213.5364181560101713 ) ) ;
#10629=CARTESIAN_POINT ( 'NONE',  ( 4.519237161608626430, -292.3008710849157978, -210.4681249279509530 ) ) ;
#10631=CARTESIAN_POINT ( 'NONE',  ( 16.47886361846065029, -289.3888988437019520, -325.0686621205390452 ) ) ;
#10632=CARTESIAN_POINT ( 'NONE',  ( -105.6124570289506863, -279.5537901636736819, -244.0850950118223182 ) ) ;
#10633=CARTESIAN_POINT ( 'NONE',  ( -113.6371032447908931, -295.3748110933260591, -278.1395479345970898 ) ) ;
#10634=CARTESIAN_POINT ( 'NONE',  ( -54.94933603908506825, -286.4828998665522590, -195.5060316898160977 ) ) ;
#10635=CARTESIAN_POINT ( 'NONE',  ( -2.236336455902808051, -286.8371787043939207, -201.8382845890868680 ) ) ;
#10636=CARTESIAN_POINT ( 'NONE',  ( -93.43558888736643553, -284.2222558878954146, -317.1111247282262866 ) ) ;
#10637=CARTESIAN_POINT ( 'NONE',  ( -90.47616956948971279, -230.2765260022941902, -347.7368331188851016 ) ) ;
#10638=CARTESIAN_POINT ( 'NONE',  ( 187.9667495628914082, 271.0942837926032780, -138.8879291161683511 ) ) ;
#10639=CARTESIAN_POINT ( 'NONE',  ( 120.7416490522416126, 147.9237423001410434, -260.2612779276005313 ) ) ;
#10640=CARTESIAN_POINT ( 'NONE',  ( -83.11573335683996788, -276.8943094913005325, -327.4994347394787724 ) ) ;
#10641=CARTESIAN_POINT ( 'NONE',  ( -21.59999097431463255, -275.7660290891985824, -342.0123831557603467 ) ) ;
#10642=CARTESIAN_POINT ( 'NONE',  ( -70.69668826749686730, -297.1316070035990720, -201.0287902427111817 ) ) ;
#10643=CARTESIAN_POINT ( 'NONE',  ( 194.5757784920336064, 275.7176583187329015, -124.3598809796911411 ) ) ;
#10644=CARTESIAN_POINT ( 'NONE',  ( -99.26056766693801592, -276.6367058874288318, -315.3206028598488615 ) ) ;
#10645=CARTESIAN_POINT ( 'NONE',  ( -69.95742892865899876, -275.3766284193590081, -203.9217602844356065 ) ) ;
#10648=CARTESIAN_POINT ( 'NONE',  ( -110.4295239542293956, -291.0694758379698328, -268.4664138691078392 ) ) ;
#10649=CARTESIAN_POINT ( 'NONE',  ( -89.50619830964393486, -298.1424108984377881, -213.8707378199553659 ) ) ;
#10650=CARTESIAN_POINT ( 'NONE',  ( -70.70802993305116502, -298.1161419401509534, -201.0342477304540125 ) ) ;
#10651=CARTESIAN_POINT ( 'NONE',  ( 1.571629225388392781, -294.6831277847397814, -332.1846717413249053 ) ) ;
#10654=CARTESIAN_POINT ( 'NONE',  ( -2.116939386304322657, -278.5096384412079260, -337.2081854660076488 ) ) ;
#10656=CARTESIAN_POINT ( 'NONE',  ( -21.74459379324450836, -282.3650317885534946, -345.7020575641483902 ) ) ;
#10657=CARTESIAN_POINT ( 'NONE',  ( -56.65070393972205665, -278.2483716366264161, -341.0577547131726419 ) ) ;
#10658=CARTESIAN_POINT ( 'NONE',  ( 34.25385029062328357, -277.6396244676450920, -295.9731916860246770 ) ) ;
#10659=CARTESIAN_POINT ( 'NONE',  ( -95.74572301409510544, -295.7519254657343026, -225.5706796945248698 ) ) ;
#10661=CARTESIAN_POINT ( 'NONE',  ( -87.09398087807991828, -277.9354448429132276, -323.7812505606715945 ) ) ;
#10662=CARTESIAN_POINT ( 'NONE',  ( 11.67480567098142608, -275.5152017053350733, -211.1181655909082338 ) ) ;
#10663=CARTESIAN_POINT ( 'NONE',  ( 12.08440007273762618, -287.0660263978285229, -328.7593961284276247 ) ) ;
#10665=CARTESIAN_POINT ( 'NONE',  ( -31.44343004379908990, -276.1267746473257603, -195.5804676336160810 ) ) ;
#10666=CARTESIAN_POINT ( 'NONE',  ( 19.42718347035934201, -274.8267114237044666, -321.5265647942315468 ) ) ;
#10668=CARTESIAN_POINT ( 'NONE',  ( -23.76521645923465798, -288.0715237638189592, -342.3036859560483549 ) ) ;
#10669=CARTESIAN_POINT ( 'NONE',  ( -65.83187507613813239, -285.0376952101303232, -198.9213382334257290 ) ) ;
#10670=CARTESIAN_POINT ( 'NONE',  ( 34.63034627907831009, -280.0173169810651075, -287.6776047824728835 ) ) ;
#10671=CARTESIAN_POINT ( 'NONE',  ( 19.79816039281242368, -280.7779916982752866, -316.7535019160187630 ) ) ;
#10672=CARTESIAN_POINT ( 'NONE',  ( -111.0343867755999412, -282.7681059504021164, -259.8396098831517520 ) ) ;
#10673=CARTESIAN_POINT ( 'NONE',  ( -97.50034916441894950, -291.9405220406471813, -315.1698539241114077 ) ) ;
#10674=CARTESIAN_POINT ( 'NONE',  ( -93.01787794354686412, -279.0799752551828874, -318.1867777227880651 ) ) ;
#10675=CARTESIAN_POINT ( 'NONE',  ( -112.7898535754452070, -271.0197564485751514, -296.3298950837670986 ) ) ;
#10676=CARTESIAN_POINT ( 'NONE',  ( 38.72911144306201692, -280.0185624848528505, -275.6261384257576879 ) ) ;
#10677=CARTESIAN_POINT ( 'NONE',  ( 37.25082834313838021, -295.6587166317874562, -278.6479071567125629 ) ) ;
#10678=CARTESIAN_POINT ( 'NONE',  ( -42.34070906176545179, -278.2297853337713605, -194.5390636451637363 ) ) ;
#10679=CARTESIAN_POINT ( 'NONE',  ( -70.89690419347613215, -285.4939989572815193, -337.6223751132505981 ) ) ;
#10681=CARTESIAN_POINT ( 'NONE',  ( -112.8118093759850495, -292.4253476089225501, -274.0457896863701990 ) ) ;
#10682=CARTESIAN_POINT ( 'NONE',  ( 7.458099028678516262, -285.8428295890606137, -207.8685272506551485 ) ) ;
#10683=CARTESIAN_POINT ( 'NONE',  ( -36.17324510314739427, -290.4668764990971113, -196.5577527448681394 ) ) ;
#10685=CARTESIAN_POINT ( 'NONE',  ( 21.21980197018436343, -274.8568333750899342, -314.7660045527009061 ) ) ;
#10686=CARTESIAN_POINT ( 'NONE',  ( -67.82370301165823889, -293.5960963828719628, -338.0634103063202360 ) ) ;
#10689=CARTESIAN_POINT ( 'NONE',  ( 14.97700674828470291, -291.2534639919134634, -214.7416269469087240 ) ) ;
#10690=CARTESIAN_POINT ( 'NONE',  ( -109.7174840115487626, -286.3405579096062183, -255.9324546953190520 ) ) ;
#10691=CARTESIAN_POINT ( 'NONE',  ( -15.26831779957030832, -287.0102001816077859, -343.1261007486804147 ) ) ;
#10692=CARTESIAN_POINT ( 'NONE',  ( -37.29860563804250972, -287.4779394910289056, -196.7593603668306343 ) ) ;
#10694=CARTESIAN_POINT ( 'NONE',  ( 35.84160461819834609, -288.3278303625476724, -268.2977278835032280 ) ) ;
#10695=CARTESIAN_POINT ( 'NONE',  ( 7.844060603488878236, -294.6453547245783398, -209.9913339980942339 ) ) ;
#10697=CARTESIAN_POINT ( 'NONE',  ( -109.3029134487697434, -276.3348439394575280, -293.5709773389618817 ) ) ;
#10698=CARTESIAN_POINT ( 'NONE',  ( -28.59922168061781278, -277.2775703214923055, -346.8954827347368450 ) ) ;
#10699=CARTESIAN_POINT ( 'NONE',  ( 0.9910615056859225502, -290.6389232828684612, -205.1866954115612600 ) ) ;
#10700=CARTESIAN_POINT ( 'NONE',  ( -112.7175445974691428, -278.7496880259101886, -254.5659702265035094 ) ) ;
#10701=CARTESIAN_POINT ( 'NONE',  ( -50.26287168460399357, -299.8662985259423408, -196.8431601382698091 ) ) ;
#10702=CARTESIAN_POINT ( 'NONE',  ( -8.706848857124272811, -284.4266351327742086, -201.0287989254448746 ) ) ;
#10704=CARTESIAN_POINT ( 'NONE',  ( -111.6280718298464620, -276.6883823284501318, -270.6190943611029525 ) ) ;
#10706=CARTESIAN_POINT ( 'NONE',  ( 10.20451192151873165, -280.3967150932363666, -328.4313936975426600 ) ) ;
#10709=CARTESIAN_POINT ( 'NONE',  ( 0.6845688316304823218, -275.0350042511108200, -336.5777569629277082 ) ) ;
#10710=CARTESIAN_POINT ( 'NONE',  ( -108.6354617769533917, -297.8277384674277641, -289.0632322392954165 ) ) ;
#10711=CARTESIAN_POINT ( 'NONE',  ( -30.25718915281167298, -281.8848392025566341, -346.7240816089750410 ) ) ;
#10712=CARTESIAN_POINT ( 'NONE',  ( -88.29804044472858493, -298.2585208316266403, -217.6893557660566216 ) ) ;
#10713=CARTESIAN_POINT ( 'NONE',  ( -65.37699570403054850, -299.0085430517990517, -199.1193739938315161 ) ) ;
#10714=CARTESIAN_POINT ( 'NONE',  ( -31.33374103302742597, -273.7968042423041197, -197.5748986713184649 ) ) ;
#10715=CARTESIAN_POINT ( 'NONE',  ( 10.09463929519419700, -294.7057653977937548, -212.2007941678915870 ) ) ;
#10716=CARTESIAN_POINT ( 'NONE',  ( 37.14495329348281416, -287.9630790946376919, -289.8736387469426745 ) ) ;
#10717=CARTESIAN_POINT ( 'NONE',  ( -38.12988750001531457, -278.1221983212080318, -194.8052250104931886 ) ) ;
#10718=CARTESIAN_POINT ( 'NONE',  ( -114.3687848332295260, -290.4105918263243211, -268.3525939512876448 ) ) ;
#10719=CARTESIAN_POINT ( 'NONE',  ( 35.23097408159468102, -286.4767709902948809, -260.1609494522082286 ) ) ;
#10720=CARTESIAN_POINT ( 'NONE',  ( -85.21628041027933875, -289.3912532301557121, -212.5613459844066426 ) ) ;
#10722=CARTESIAN_POINT ( 'NONE',  ( 198.4603912096053193, 279.4542985770845576, -127.2015713121144529 ) ) ;
#10723=CARTESIAN_POINT ( 'NONE',  ( -29.17246090628071897, -288.4534831264834907, -342.9645061414113911 ) ) ;
#10726=CARTESIAN_POINT ( 'NONE',  ( -91.74471522434500059, -286.2405678004562901, -216.2027191778190343 ) ) ;
#10727=CARTESIAN_POINT ( 'NONE',  ( -8.588195852930263996, -291.4781644400528080, -199.1848845544936637 ) ) ;
#10728=CARTESIAN_POINT ( 'NONE',  ( -7.865464708224273238, -282.0320895933588758, -200.0789643550781136 ) ) ;
#10729=CARTESIAN_POINT ( 'NONE',  ( -7.743340382072014805, -281.7471812536335847, -199.7973837385956983 ) ) ;
#10730=CARTESIAN_POINT ( 'NONE',  ( -95.11774214064784871, -283.7570283898784282, -315.0013508448441826 ) ) ;
#10731=CARTESIAN_POINT ( 'NONE',  ( 1.940068575895329328, -278.5270857289665400, -334.3122409987219044 ) ) ;
#10732=CARTESIAN_POINT ( 'NONE',  ( -82.97057633259714748, -297.4472980442525341, -208.2706356750579744 ) ) ;
#10733=CARTESIAN_POINT ( 'NONE',  ( -92.39863832334661709, -274.5581645179314023, -221.6787080653439546 ) ) ;
#10734=CARTESIAN_POINT ( 'NONE',  ( 32.37336996393432997, -291.2238401860857380, -243.6842403021568089 ) ) ;
#10735=CARTESIAN_POINT ( 'NONE',  ( -94.91467594722058720, -271.9860455555678982, -224.8365865566790944 ) ) ;
#10738=CARTESIAN_POINT ( 'NONE',  ( -109.4291553198203815, -286.7126552196176590, -251.7946696248425837 ) ) ;
#10739=CARTESIAN_POINT ( 'NONE',  ( 0.4004077071593539761, -295.6412293317794706, -337.1371981409969862 ) ) ;
#10740=CARTESIAN_POINT ( 'NONE',  ( -103.5813378733372048, -285.6219723232832166, -239.3185583255447284 ) ) ;
#10741=CARTESIAN_POINT ( 'NONE',  ( -45.63614427752890634, -276.2134521006823888, -346.7292975434579603 ) ) ;
#10742=CARTESIAN_POINT ( 'NONE',  ( -11.19572241598899431, -293.0353898945530204, -197.9884879881219604 ) ) ;
#10743=CARTESIAN_POINT ( 'NONE',  ( 37.34335100084359738, -285.5287685181241386, -257.5391240864649376 ) ) ;
#10744=CARTESIAN_POINT ( 'NONE',  ( 28.03215758393609036, -293.3524563055941030, -229.6155661232588443 ) ) ;
#10745=CARTESIAN_POINT ( 'NONE',  ( -50.75118453917053785, -289.5613363637224893, -342.1921481868440083 ) ) ;
#10748=CARTESIAN_POINT ( 'NONE',  ( -11.96379597270533246, -92.71834851594391580, -356.3861524803674570 ) ) ;
#10749=CARTESIAN_POINT ( 'NONE',  ( -100.8314115110139966, -285.5089738210984933, -312.7851289677623186 ) ) ;
#10750=CARTESIAN_POINT ( 'NONE',  ( -55.56934967048407970, -271.3380690714491266, -190.3538533559490702 ) ) ;
#10752=CARTESIAN_POINT ( 'NONE',  ( -2.292921609286411311, -281.4971299140666474, -334.7634250203108763 ) ) ;
#10753=CARTESIAN_POINT ( 'NONE',  ( -103.3912703137021083, -278.7357302904979974, -230.7201766575317095 ) ) ;
#10754=CARTESIAN_POINT ( 'NONE',  ( -27.33789394480205104, -282.1795958632827137, -196.1469801832075461 ) ) ;
#10755=CARTESIAN_POINT ( 'NONE',  ( 204.5909795363367891, 292.7457261787433254, -68.41955665847963530 ) ) ;
#10756=CARTESIAN_POINT ( 'NONE',  ( 6.571430675641973806, -281.0432031440411151, -332.9577466885220360 ) ) ;
#10757=CARTESIAN_POINT ( 'NONE',  ( 3.364626072031145831, -284.6224133318508507, -207.7924212691952448 ) ) ;
#10758=CARTESIAN_POINT ( 'NONE',  ( -70.30993356764764712, -299.3837306600277657, -201.8989415500608686 ) ) ;
#10759=CARTESIAN_POINT ( 'NONE',  ( -84.51305674767031917, -296.2144103521828242, -326.2204732505211950 ) ) ;
#10761=CARTESIAN_POINT ( 'NONE',  ( 21.39797931591046520, -291.6209156172562302, -226.1921974834140769 ) ) ;
#10762=CARTESIAN_POINT ( 'NONE',  ( -35.70535089044972921, -277.6835718867363880, -347.2548793080964060 ) ) ;
#10763=CARTESIAN_POINT ( 'NONE',  ( -34.04067943773179650, -274.0948255241699485, -197.4357913641492530 ) ) ;
#10764=CARTESIAN_POINT ( 'NONE',  ( 25.08332321250857788, -273.8797677761762088, -225.7896970097445717 ) ) ;
#10766=CARTESIAN_POINT ( 'NONE',  ( 20.52236573926490948, -272.8935817134516242, -222.6259801913265903 ) ) ;
#10767=CARTESIAN_POINT ( 'NONE',  ( -53.14948574445699592, -296.6761351236754081, -345.1729843435741145 ) ) ;
#10770=CARTESIAN_POINT ( 'NONE',  ( -100.6612366153629949, -285.1269098186397173, -307.3051617790441696 ) ) ;
#10771=CARTESIAN_POINT ( 'NONE',  ( -13.71544771838811272, -284.5097588080453193, -342.5814351326961855 ) ) ;
#10772=CARTESIAN_POINT ( 'NONE',  ( -90.82168271424853856, -283.1850622910399125, -320.1986954802123364 ) ) ;
#10773=CARTESIAN_POINT ( 'NONE',  ( 3.560745142417650388, -274.8916413858188434, -331.7893719442473639 ) ) ;
#10774=CARTESIAN_POINT ( 'NONE',  ( 19.45443789176212590, -284.0804687698538373, -318.1832037913939075 ) ) ;
#10775=CARTESIAN_POINT ( 'NONE',  ( -74.37831570381685253, -276.0341931432435558, -334.0713750799314994 ) ) ;
#10776=CARTESIAN_POINT ( 'NONE',  ( 5.345624557889809836, -275.7244538737770085, -210.6995728644445478 ) ) ;
#10778=CARTESIAN_POINT ( 'NONE',  ( -88.83083171737196437, -280.1532866199092950, -213.3257942941159797 ) ) ;
#10782=CARTESIAN_POINT ( 'NONE',  ( -109.9178383830745247, -286.1346626059899450, -292.1549054862393291 ) ) ;
#10783=CARTESIAN_POINT ( 'NONE',  ( -55.85402052730736244, -294.4936941070247371, -341.1942362067428576 ) ) ;
#10784=CARTESIAN_POINT ( 'NONE',  ( -106.4255897000815310, -289.4650977865974824, -304.2568610767687574 ) ) ;
#10785=CARTESIAN_POINT ( 'NONE',  ( 36.12742990191152614, -285.9085694237666644, -279.3199653169455132 ) ) ;
#10786=CARTESIAN_POINT ( 'NONE',  ( 31.53244297848572941, -285.7820867721393938, -244.2994724476738213 ) ) ;
#10787=CARTESIAN_POINT ( 'NONE',  ( -55.23595138817798045, -290.0586605688069994, -198.5435032715879800 ) ) ;
#10788=CARTESIAN_POINT ( 'NONE',  ( -70.37998880068430196, -284.7027265713878137, -335.9160135341392106 ) ) ;
#10789=CARTESIAN_POINT ( 'NONE',  ( -23.33797735764125747, -274.8730716069424602, -344.0949378249958954 ) ) ;
#10790=CARTESIAN_POINT ( 'NONE',  ( -26.28101928264467801, -287.3134790043345106, -345.7541001039717230 ) ) ;
#10791=CARTESIAN_POINT ( 'NONE',  ( -4.391616713646087078, -288.4865236114843583, -202.9726973185919405 ) ) ;
#10792=CARTESIAN_POINT ( 'NONE',  ( 37.16158397909956079, -285.4243330105232985, -260.3967272066142300 ) ) ;
#10794=CARTESIAN_POINT ( 'NONE',  ( -21.32511947821312503, -283.7830491607134604, -341.8757210210810058 ) ) ;
#10795=CARTESIAN_POINT ( 'NONE',  ( -36.09117268585716687, -291.0366967902178317, -345.5301837841675479 ) ) ;
#10798=CARTESIAN_POINT ( 'NONE',  ( -110.5669710796004352, -298.2340350577171648, -289.0512529991289625 ) ) ;
#10799=CARTESIAN_POINT ( 'NONE',  ( -73.06037851496463986, -277.5785202567057581, -204.4128301731372801 ) ) ;
#10800=CARTESIAN_POINT ( 'NONE',  ( 36.13556649406574905, -292.4664911062952228, -247.8833487367799080 ) ) ;
#10801=CARTESIAN_POINT ( 'NONE',  ( -99.10605657217521980, -295.5068704226681007, -229.8755504850865066 ) ) ;
#10802=CARTESIAN_POINT ( 'NONE',  ( 36.05760788783123871, -280.2856208235211852, -274.0739416475793746 ) ) ;
#10803=CARTESIAN_POINT ( 'NONE',  ( -27.06770729667313091, -272.2634707912317253, -196.5816123494329020 ) ) ;
#10804=CARTESIAN_POINT ( 'NONE',  ( -12.82807071576416291, -296.0420645993426660, -339.6991220518505088 ) ) ;
#10806=CARTESIAN_POINT ( 'NONE',  ( -36.88240502880744032, -296.5376888537812761, -194.0545626491387168 ) ) ;
#10807=CARTESIAN_POINT ( 'NONE',  ( 27.23279826132012005, -292.3239484210758405, -310.5112463240487841 ) ) ;
#10808=CARTESIAN_POINT ( 'NONE',  ( -19.95037179710934794, -293.7052263745741243, -198.8037682244255393 ) ) ;
#10811=CARTESIAN_POINT ( 'NONE',  ( 29.64199254337842859, -294.7499597974837684, -299.7853706077844436 ) ) ;
#10813=CARTESIAN_POINT ( 'NONE',  ( -13.95681954484038023, -280.7703279347120997, -341.9959849197629183 ) ) ;
#10814=CARTESIAN_POINT ( 'NONE',  ( 22.93299158719334230, -294.1262432090257448, -311.6315678334925678 ) ) ;
#10815=CARTESIAN_POINT ( 'NONE',  ( 4.545697659568949334, -282.5040189849777903, -335.0340880772603782 ) ) ;
#10816=CARTESIAN_POINT ( 'NONE',  ( -24.54127771001219571, -282.5599228706585677, -346.3223557989367123 ) ) ;
#10817=CARTESIAN_POINT ( 'NONE',  ( -108.3018575485358355, -288.8598716072951902, -246.5980271723541080 ) ) ;
#10820=CARTESIAN_POINT ( 'NONE',  ( 0.5074842209121356307, -281.0371973676857920, -336.6343954390261501 ) ) ;
#10821=CARTESIAN_POINT ( 'NONE',  ( 10.02618436395603574, -287.3373294296103495, -330.7426462517533992 ) ) ;
#10823=CARTESIAN_POINT ( 'NONE',  ( -93.68005681340099500, -297.4819076684323704, -318.0506995621724400 ) ) ;
#10824=CARTESIAN_POINT ( 'NONE',  ( -2.973746193010138761, -278.0322934168884217, -338.6211980143785354 ) ) ;
#10825=CARTESIAN_POINT ( 'NONE',  ( -96.42031208133099085, -278.8193177483025238, -227.4448611967359000 ) ) ;
#10826=CARTESIAN_POINT ( 'NONE',  ( -0.8057297394032891802, -292.6904119392962116, -202.5811587595218839 ) ) ;
#10827=CARTESIAN_POINT ( 'NONE',  ( -107.9659192529368994, -282.2838443460601070, -297.3684241014060490 ) ) ;
#10828=CARTESIAN_POINT ( 'NONE',  ( -100.4012304306613430, -280.0042594209836011, -311.0575154519202670 ) ) ;
#10829=CARTESIAN_POINT ( 'NONE',  ( 35.53072565946914096, -292.5086950613564341, -262.5888175399512647 ) ) ;
#10830=CARTESIAN_POINT ( 'NONE',  ( -92.18247048047500414, -295.2687883225282803, -219.1239768872219713 ) ) ;
#10833=CARTESIAN_POINT ( 'NONE',  ( 19.73791417178628649, -293.7036940799531521, -315.9870467865972046 ) ) ;
#10835=CARTESIAN_POINT ( 'NONE',  ( -21.33282851196157992, -283.7666405000204009, -200.3683826091710216 ) ) ;
#10836=CARTESIAN_POINT ( 'NONE',  ( -30.49857286833661973, -297.1946158561257221, -193.5974729951946927 ) ) ;
#10837=CARTESIAN_POINT ( 'NONE',  ( 29.69134896089387965, -288.3853977817511236, -233.3748410405109723 ) ) ;
#10838=CARTESIAN_POINT ( 'NONE',  ( 33.70059731441377693, -287.6070069351031293, -287.1537347717867874 ) ) ;
#10839=CARTESIAN_POINT ( 'NONE',  ( -109.7206254024223284, -279.8903384900612537, -284.2840710866177005 ) ) ;
#10840=CARTESIAN_POINT ( 'NONE',  ( -44.69171579865019339, -299.7181538927221709, -196.6625565816640631 ) ) ;
#10841=CARTESIAN_POINT ( 'NONE',  ( -106.6441851294882071, -277.0254538375502875, -294.6875665123658337 ) ) ;
#10843=CARTESIAN_POINT ( 'NONE',  ( -35.82440477963562842, -297.7373833247249877, -193.3823448134014029 ) ) ;
#10844=CARTESIAN_POINT ( 'NONE',  ( -95.20855611956925202, -291.8227431082970611, -317.1878323606499634 ) ) ;
#10845=CARTESIAN_POINT ( 'NONE',  ( 19.76548821246756660, -294.4617080423584525, -219.8913421643067636 ) ) ;
#10846=CARTESIAN_POINT ( 'NONE',  ( -113.7095423085087020, -274.0181020978040465, -270.3797830366729045 ) ) ;
#10847=CARTESIAN_POINT ( 'NONE',  ( -109.0370756374908154, -291.0147268003102567, -284.6962616743735452 ) ) ;
#10849=CARTESIAN_POINT ( 'NONE',  ( -47.55307952463697063, -290.0633954504446592, -195.2346694022549514 ) ) ;
#10850=CARTESIAN_POINT ( 'NONE',  ( -23.36885445191075661, -298.5558941747436847, -193.3814952637580404 ) ) ;
#10852=CARTESIAN_POINT ( 'NONE',  ( -37.14529423159790866, -297.7214037756789367, -197.3371356321057419 ) ) ;
#10856=CARTESIAN_POINT ( 'NONE',  ( -107.0896973209595302, -291.6722254895928472, -301.4413591983838501 ) ) ;
#10857=CARTESIAN_POINT ( 'NONE',  ( 13.84574458161073096, -296.9090924074130839, -334.4957818155094174 ) ) ;
#10858=CARTESIAN_POINT ( 'NONE',  ( -97.24852301069863358, -287.1663516274887229, -225.5147022773129493 ) ) ;
#10859=CARTESIAN_POINT ( 'NONE',  ( 31.88014990409208949, -273.1786910828441250, -241.7931953196790289 ) ) ;
#10860=CARTESIAN_POINT ( 'NONE',  ( -88.33724893539921652, -275.2516448583933766, -216.0616695809800092 ) ) ;
#10862=CARTESIAN_POINT ( 'NONE',  ( 21.33273617967000746, -290.9985811533958326, -224.5297248194005135 ) ) ;
#10863=CARTESIAN_POINT ( 'NONE',  ( -38.50189744499982680, -278.9269643535832870, -346.1170380564475408 ) ) ;
#10864=CARTESIAN_POINT ( 'NONE',  ( -65.36243024302865479, -282.7769334377372275, -337.8931141727234149 ) ) ;
#10865=CARTESIAN_POINT ( 'NONE',  ( -86.88498033598381198, -278.8022031872486650, -328.9707981743637788 ) ) ;
#10866=CARTESIAN_POINT ( 'NONE',  ( -5.097092581668983158, -279.2621815445925222, -200.8751913184327123 ) ) ;
#10867=CARTESIAN_POINT ( 'NONE',  ( -104.0266749948802669, -253.6705548287846455, -324.5544463287839108 ) ) ;
#10868=CARTESIAN_POINT ( 'NONE',  ( 21.66229184770098115, -275.8308804817950772, -221.2556280171031347 ) ) ;
#10870=CARTESIAN_POINT ( 'NONE',  ( -68.57811553201872812, -275.1692114448493953, -200.7264935143020068 ) ) ;
#10871=CARTESIAN_POINT ( 'NONE',  ( -37.37352853689063181, -276.5519495502701375, -200.3611179825600459 ) ) ;
#10875=CARTESIAN_POINT ( 'NONE',  ( -34.55252550378722987, -290.0960972906104871, -343.6669433406570988 ) ) ;
#10876=CARTESIAN_POINT ( 'NONE',  ( 38.68889953193243514, -289.3268948880912603, -271.5132555848437050 ) ) ;
#10877=CARTESIAN_POINT ( 'NONE',  ( -103.6452925671211034, -290.3157169835753848, -239.5759543886024687 ) ) ;
#10878=CARTESIAN_POINT ( 'NONE',  ( 27.08965273544284003, -286.5069571964024817, -228.3120077498088847 ) ) ;
#10880=CARTESIAN_POINT ( 'NONE',  ( 36.36388678617412040, -280.0007123266805706, -274.0929902922406427 ) ) ;
#10881=CARTESIAN_POINT ( 'NONE',  ( 8.765337633554176833, -290.2726655128453785, -328.5419270717350742 ) ) ;
#10882=CARTESIAN_POINT ( 'NONE',  ( -56.51778961428590975, -281.7837064650937577, -341.5157758952734639 ) ) ;
#10883=CARTESIAN_POINT ( 'NONE',  ( -68.74913522007797440, -280.9455571570364327, -203.9170324626630872 ) ) ;
#10884=CARTESIAN_POINT ( 'NONE',  ( 39.34188165271749682, -288.4364396345058026, -265.8203297771192410 ) ) ;
#10885=CARTESIAN_POINT ( 'NONE',  ( -83.04036938952030766, -278.1892808830866102, -327.4316655560248819 ) ) ;
#10886=CARTESIAN_POINT ( 'NONE',  ( -111.2456412186606514, -289.6013897656955010, -250.1565755494168286 ) ) ;
#10887=CARTESIAN_POINT ( 'NONE',  ( -104.2713272462240468, -284.8629556578851520, -308.2125189117822970 ) ) ;
#10888=CARTESIAN_POINT ( 'NONE',  ( -33.73648894178771940, -286.5887254025682296, -193.5071697713474350 ) ) ;
#10889=CARTESIAN_POINT ( 'NONE',  ( -70.21302376918448829, -283.6644988937621292, -335.5554315235995659 ) ) ;
#10892=CARTESIAN_POINT ( 'NONE',  ( -111.9597024112458570, -292.5794805507978822, -257.2287451113072621 ) ) ;
#10893=CARTESIAN_POINT ( 'NONE',  ( 29.05601480467808528, -291.7399915758287534, -232.3526751914484691 ) ) ;
#10894=CARTESIAN_POINT ( 'NONE',  ( -31.30841593742026419, -273.1889315191523337, -197.3620731682969449 ) ) ;
#10895=CARTESIAN_POINT ( 'NONE',  ( -72.03548057987100606, -294.8474461953565537, -338.9880397041938522 ) ) ;
#10896=CARTESIAN_POINT ( 'NONE',  ( -90.30125678704624193, -289.7656129742889561, -219.1166733008099925 ) ) ;
#10897=CARTESIAN_POINT ( 'NONE',  ( -68.97045614702022931, -293.7136667199707176, -337.2898813892948624 ) ) ;
#10898=CARTESIAN_POINT ( 'NONE',  ( -7.120697760712635827, -293.6628054910511878, -203.4744861206333724 ) ) ;
#10900=CARTESIAN_POINT ( 'NONE',  ( 37.87703502512747633, -291.5516737012878252, -270.3365989762054369 ) ) ;
#10901=CARTESIAN_POINT ( 'NONE',  ( -78.60353246568196539, -297.6075134645395224, -333.0516871339069098 ) ) ;
#10902=CARTESIAN_POINT ( 'NONE',  ( 34.22339099837354581, -288.2889165938020142, -254.8097135135828921 ) ) ;
#10903=CARTESIAN_POINT ( 'NONE',  ( -25.99226979892631206, -278.8881998667927178, -344.8567368587943633 ) ) ;
#10904=CARTESIAN_POINT ( 'NONE',  ( -45.62202854961023490, -275.9496708821050674, -346.5679896372945450 ) ) ;
#10905=CARTESIAN_POINT ( 'NONE',  ( -93.53765840327440628, -296.4659230409811244, -217.8795776110415829 ) ) ;
#10906=CARTESIAN_POINT ( 'NONE',  ( 1.382771120973315337, -274.7673902280189964, -333.4958028998477744 ) ) ;
#10907=CARTESIAN_POINT ( 'NONE',  ( -100.6803746712757288, -277.1620261672334209, -231.1536718745393273 ) ) ;
#10908=CARTESIAN_POINT ( 'NONE',  ( -109.9111147165462228, -276.6548180003418906, -293.7716438872411686 ) ) ;
#10911=CARTESIAN_POINT ( 'NONE',  ( -87.40915018039754614, -273.9831083231292723, -217.0269643228989764 ) ) ;
#10914=CARTESIAN_POINT ( 'NONE',  ( -20.88079449138717791, -286.8621482966319149, -343.9499475225034075 ) ) ;
#10915=CARTESIAN_POINT ( 'NONE',  ( -21.93195891545083853, -274.0884831370159986, -199.0060909680411783 ) ) ;
#10917=CARTESIAN_POINT ( 'NONE',  ( 37.37682736240206083, -287.3193898071705235, -251.7562355681538975 ) ) ;
#10918=CARTESIAN_POINT ( 'NONE',  ( -112.5083667949886888, -274.5519907589103354, -270.3865271280112097 ) ) ;
#10919=CARTESIAN_POINT ( 'NONE',  ( -98.70085006719020271, -293.9693470209815587, -313.1989884521789804 ) ) ;
#10921=CARTESIAN_POINT ( 'NONE',  ( 17.70344643396533613, -281.4866221237117543, -324.0486128710462026 ) ) ;
#10923=CARTESIAN_POINT ( 'NONE',  ( 10.92051741093306205, -278.7192061292386711, -212.8853281000835125 ) ) ;
#10925=CARTESIAN_POINT ( 'NONE',  ( -109.3311876663043307, -289.1585381048878958, -284.7308602091442822 ) ) ;
#10928=CARTESIAN_POINT ( 'NONE',  ( -111.2431445606223548, -288.7200106620329620, -257.2754408121874121 ) ) ;
#10929=CARTESIAN_POINT ( 'NONE',  ( 5.564858526132587357, -276.1648335446911346, -210.3836622949784498 ) ) ;
#10930=CARTESIAN_POINT ( 'NONE',  ( 13.30392837838768472, -283.7856787407495176, -327.6471775522419989 ) ) ;
#10931=CARTESIAN_POINT ( 'NONE',  ( -51.46703495452751298, -295.8926230805512319, -196.2884743318714413 ) ) ;
#10932=CARTESIAN_POINT ( 'NONE',  ( -26.74277571119780816, -282.9137202105658275, -342.6388864808363905 ) ) ;
#10933=CARTESIAN_POINT ( 'NONE',  ( -5.065874897012928813, -275.9108686779624122, -204.2136374346252978 ) ) ;
#10934=CARTESIAN_POINT ( 'NONE',  ( -2.846534649821085949, -275.3233428741677926, -205.8422425588160820 ) ) ;
#10936=CARTESIAN_POINT ( 'NONE',  ( -68.33606214928872191, -285.4594106713332735, -338.6712030926112789 ) ) ;
#10937=CARTESIAN_POINT ( 'NONE',  ( -37.81203744875236339, -297.1048641811096331, -197.1273332126014566 ) ) ;
#10940=CARTESIAN_POINT ( 'NONE',  ( 39.44122556016269243, -293.3132138825386050, -264.5833738515132154 ) ) ;
#10941=CARTESIAN_POINT ( 'NONE',  ( -97.22656306484043398, -285.9207346792924227, -314.9217507922982691 ) ) ;
#10944=CARTESIAN_POINT ( 'NONE',  ( 36.60358173371529489, -278.6237833571632905, -234.7871824221999191 ) ) ;
#10945=CARTESIAN_POINT ( 'NONE',  ( -84.77474732016597159, -276.8840595240507696, -330.8792488849715596 ) ) ;
#10946=CARTESIAN_POINT ( 'NONE',  ( -111.4890281604978668, -288.7293136408266605, -287.9844273774644421 ) ) ;
#10947=CARTESIAN_POINT ( 'NONE',  ( -56.48049038906741970, -284.8234610527591144, -341.5258175041921618 ) ) ;
#10948=CARTESIAN_POINT ( 'NONE',  ( -39.16050599114966246, -278.8354312450923089, -344.3521036569139255 ) ) ;
#10949=CARTESIAN_POINT ( 'NONE',  ( -93.49911713459866291, -286.6889984507919280, -218.4670415465290034 ) ) ;
#10950=CARTESIAN_POINT ( 'NONE',  ( -24.55992040486605887, -282.2154531726777691, -196.4582983260262381 ) ) ;
#10951=CARTESIAN_POINT ( 'NONE',  ( 26.92939223182577280, -275.1611961526215850, -227.9556149037361195 ) ) ;
#10952=CARTESIAN_POINT ( 'NONE',  ( -31.45238450712145450, -276.8131841377852425, -347.1881899096321717 ) ) ;
#10953=CARTESIAN_POINT ( 'NONE',  ( -99.93106445781967295, -297.9242670308082666, -310.7529661689855516 ) ) ;
#10955=CARTESIAN_POINT ( 'NONE',  ( -106.6662871844225293, -281.4805209788417528, -237.0123917617630980 ) ) ;
#10956=CARTESIAN_POINT ( 'NONE',  ( -109.1369972974880937, -271.1099784194080371, -245.4731828104865201 ) ) ;
#10957=CARTESIAN_POINT ( 'NONE',  ( -16.36919670121143611, -276.2814407686956315, -340.4009013751984867 ) ) ;
#10958=CARTESIAN_POINT ( 'NONE',  ( -21.45220796181182621, -275.4566289245137227, -195.4242595204761983 ) ) ;
#10959=CARTESIAN_POINT ( 'NONE',  ( 35.99716102564403997, -289.1777284591159969, -260.0183744527114413 ) ) ;
#10960=CARTESIAN_POINT ( 'NONE',  ( -44.70923719324815693, -296.6637711608207155, -346.3642052802466651 ) ) ;
#10961=CARTESIAN_POINT ( 'NONE',  ( -33.43963587920578817, -296.2091580762302669, -346.8776506496019465 ) ) ;
#10962=CARTESIAN_POINT ( 'NONE',  ( -104.0552475132521550, -293.0027907728751870, -236.3445484442329700 ) ) ;
#10963=CARTESIAN_POINT ( 'NONE',  ( -1.055344631209611528, -278.5348183071635617, -204.9139726459793565 ) ) ;
#10964=CARTESIAN_POINT ( 'NONE',  ( -3.718603246501502646, -282.4194396576424992, -203.9330890450153788 ) ) ;
#10965=CARTESIAN_POINT ( 'NONE',  ( -89.10994746790565557, -295.3975757147995864, -216.7974677063391482 ) ) ;
#10966=CARTESIAN_POINT ( 'NONE',  ( -58.12480224572666998, -285.1781700703280080, -343.2742699700966114 ) ) ;
#10967=CARTESIAN_POINT ( 'NONE',  ( 24.49172460557148412, -287.0147056594360038, -309.7419973420132919 ) ) ;
#10968=CARTESIAN_POINT ( 'NONE',  ( -20.36879062156694786, -109.3229610787347923, -362.1159644462802021 ) ) ;
#10970=CARTESIAN_POINT ( 'NONE',  ( 35.70163485141603132, -287.1918994139536494, -268.3161009710789813 ) ) ;
#10972=CARTESIAN_POINT ( 'NONE',  ( -33.06219580151827131, -284.0791327376361437, -346.9455939830428974 ) ) ;
#10973=CARTESIAN_POINT ( 'NONE',  ( -56.87135073797514195, -274.1266875804957408, -199.9473149587551291 ) ) ;
#10974=CARTESIAN_POINT ( 'NONE',  ( -1.143572649972678601, -285.3165631670063931, -202.8503463500382225 ) ) ;
#10975=CARTESIAN_POINT ( 'NONE',  ( -6.336425542486779250, -281.3908171536571672, -200.1222997126138807 ) ) ;
#10977=CARTESIAN_POINT ( 'NONE',  ( -113.3550901977310730, -280.1639160325332796, -263.0993373856484823 ) ) ;
#10978=CARTESIAN_POINT ( 'NONE',  ( 28.28919821757781961, -282.4123239606552147, -310.6906093150817014 ) ) ;
#10979=CARTESIAN_POINT ( 'NONE',  ( -6.941161984400256557, -289.9809262143061233, -207.3071070584150277 ) ) ;
#10980=CARTESIAN_POINT ( 'NONE',  ( 139.6957795963261333, 180.2233390436421985, -241.5434084867537763 ) ) ;
#10983=CARTESIAN_POINT ( 'NONE',  ( 23.98249658564035869, -278.1367644760755979, -313.3380138231381693 ) ) ;
#10984=CARTESIAN_POINT ( 'NONE',  ( 202.6185701365793363, 295.9433668349635127, -68.63232107392525450 ) ) ;
#10985=CARTESIAN_POINT ( 'NONE',  ( 34.70767268040145836, -279.3196168398559962, -250.7997294482875361 ) ) ;
#10986=CARTESIAN_POINT ( 'NONE',  ( 25.68394968003943291, -295.8789684273773446, -312.8080434303172410 ) ) ;
#10987=CARTESIAN_POINT ( 'NONE',  ( -61.05406336697056702, -294.7167022270934922, -339.5640031186309784 ) ) ;
#10988=CARTESIAN_POINT ( 'NONE',  ( -7.208520942112449426, -291.9445882052895058, -199.5547283942408114 ) ) ;
#10989=CARTESIAN_POINT ( 'NONE',  ( -110.6395504404451202, -271.5021484970271217, -270.3477489206637756 ) ) ;
#10991=CARTESIAN_POINT ( 'NONE',  ( -113.5317549249391931, -295.2082840836710034, -263.9020585142498589 ) ) ;
#10992=CARTESIAN_POINT ( 'NONE',  ( 6.301493406326240887, -286.8486100140940493, -329.9370774783134266 ) ) ;
#10993=CARTESIAN_POINT ( 'NONE',  ( 36.76614841840203241, -295.3457196071952353, -265.2073783910465750 ) ) ;
#10994=CARTESIAN_POINT ( 'NONE',  ( -109.6813983477632490, -286.0382018756369575, -257.3205931007504432 ) ) ;
#10996=CARTESIAN_POINT ( 'NONE',  ( 35.26778301244063840, -294.8101879553623803, -295.4376004276389267 ) ) ;
#10998=CARTESIAN_POINT ( 'NONE',  ( -104.1670597106370053, -284.6473490094984982, -299.8968549486609163 ) ) ;
#10999=CARTESIAN_POINT ( 'NONE',  ( -111.8844013291345192, -295.5689325182196399, -252.7147467386035089 ) ) ;
#11000=CARTESIAN_POINT ( 'NONE',  ( -89.37461083492657110, -290.5658807097030376, -326.9007945244755433 ) ) ;
#11001=CARTESIAN_POINT ( 'NONE',  ( -112.8657572861379776, -291.2291570634452569, -255.6076462779012672 ) ) ;
#11002=CARTESIAN_POINT ( 'NONE',  ( -68.75605496183426624, -289.6437065493519754, -336.2560215405648592 ) ) ;
#11005=CARTESIAN_POINT ( 'NONE',  ( -102.7948592003603068, -298.9183566516531414, -232.0976227465491206 ) ) ;
#11006=CARTESIAN_POINT ( 'NONE',  ( -41.15755585938099870, -272.8001929367039224, -193.8012977609677705 ) ) ;
#11008=CARTESIAN_POINT ( 'NONE',  ( -6.659937873120455265, -279.5238850640776604, -203.8490222498963931 ) ) ;
#11009=CARTESIAN_POINT ( 'NONE',  ( -7.708479792108360762, -273.9377827044723404, -199.3017526767342815 ) ) ;
#11010=CARTESIAN_POINT ( 'NONE',  ( -105.6114186778319066, -294.6638368010980003, -298.1091499861007605 ) ) ;
#11011=CARTESIAN_POINT ( 'NONE',  ( 17.45871661260689223, -278.1191088163350855, -320.4578222363978739 ) ) ;
#11012=CARTESIAN_POINT ( 'NONE',  ( 23.30336918773956612, -273.1038502388787492, -227.5250752061944013 ) ) ;
#11013=CARTESIAN_POINT ( 'NONE',  ( -68.22853613027979236, -298.8423152017647340, -203.7655948570242970 ) ) ;
#11014=CARTESIAN_POINT ( 'NONE',  ( -110.4060775363904838, -297.5453956666506201, -276.9410109938169171 ) ) ;
#11015=CARTESIAN_POINT ( 'NONE',  ( 144.7857639756989272, -299.5541904835127980, -197.2582414438974183 ) ) ;
#11016=CARTESIAN_POINT ( 'NONE',  ( -110.4421046932612569, -297.8790715365221899, -291.9192175517947021 ) ) ;
#11017=CARTESIAN_POINT ( 'NONE',  ( 28.79935195122864400, -296.8780820938325746, -195.2169294587867796 ) ) ;
#11018=CARTESIAN_POINT ( 'NONE',  ( 25.88497798491060919, -294.7062408111802370, -307.0528042718527786 ) ) ;
#11019=CARTESIAN_POINT ( 'NONE',  ( 26.75664534524298332, -291.6348076457171601, -234.1076558627702013 ) ) ;
#11021=CARTESIAN_POINT ( 'NONE',  ( 37.18070276567564747, -276.2840839297336402, -289.4906336686852910 ) ) ;
#11022=CARTESIAN_POINT ( 'NONE',  ( -49.96174262937216781, -298.2199525940888520, -198.4387847754279051 ) ) ;
#11024=CARTESIAN_POINT ( 'NONE',  ( 35.39070111244882355, -283.2792772165214501, -250.6042633343988939 ) ) ;
#11025=CARTESIAN_POINT ( 'NONE',  ( -88.00757297697549575, -282.4279933527611774, -327.7578456336591444 ) ) ;
#11027=CARTESIAN_POINT ( 'NONE',  ( -87.03565260565629558, -277.0713971588913296, -329.1148982752972074 ) ) ;
#11029=CARTESIAN_POINT ( 'NONE',  ( -71.49329828238441564, -282.7126387187799992, -335.0625095507746778 ) ) ;
#11030=CARTESIAN_POINT ( 'NONE',  ( -99.90764157670690793, -281.9892592117703884, -312.1142658533706253 ) ) ;
#11031=ADVANCED_FACE ( 'NONE', ( #40026 ), #23243, .T. ) ;
#11032=CARTESIAN_POINT ( 'NONE',  ( 35.96690450626989843, -274.0355544208524066, -263.3827790019315671 ) ) ;
#11033=CARTESIAN_POINT ( 'NONE',  ( -104.6145755453458293, -280.1136154768362871, -303.6337203406936851 ) ) ;
#11036=CARTESIAN_POINT ( 'NONE',  ( -93.54132735638877705, -271.6595100805591301, -218.8827261971229916 ) ) ;
#11037=CARTESIAN_POINT ( 'NONE',  ( -103.3531063362100184, -280.0757008758207576, -306.3127893519672966 ) ) ;
#11039=CARTESIAN_POINT ( 'NONE',  ( -103.1506025912072460, -285.9800972611657812, -307.5952228160468849 ) ) ;
#11041=CARTESIAN_POINT ( 'NONE',  ( 31.49988911538259018, -285.1611304524824959, -240.4689079486662706 ) ) ;
#11043=CARTESIAN_POINT ( 'NONE',  ( -86.76863518983608969, -294.5530777084238139, -324.6207585483201115 ) ) ;
#11044=CARTESIAN_POINT ( 'NONE',  ( -29.05842763463842005, -287.0856349043655769, -344.1327444805640994 ) ) ;
#11046=CARTESIAN_POINT ( 'NONE',  ( -101.5974894090540204, -295.0712285570374434, -231.5795083821487879 ) ) ;
#11047=CARTESIAN_POINT ( 'NONE',  ( -49.21755219762061273, -284.3834541991189440, -194.9310016894561670 ) ) ;
#11048=CARTESIAN_POINT ( 'NONE',  ( 29.69088422181411957, -282.7388465408901652, -239.3668416304933260 ) ) ;
#11049=CARTESIAN_POINT ( 'NONE',  ( -8.445278346757712384, -280.9190452645461278, -340.6947165030421161 ) ) ;
#11050=CARTESIAN_POINT ( 'NONE',  ( -94.95056600423031057, -289.9202355592743743, -315.2167747613553388 ) ) ;
#11052=CARTESIAN_POINT ( 'NONE',  ( -96.09304980416767705, -280.5951228408779343, -226.0270613269139233 ) ) ;
#11053=CARTESIAN_POINT ( 'NONE',  ( -72.21566148290209242, -280.3810604414051113, -206.0462009982429663 ) ) ;
#11055=CARTESIAN_POINT ( 'NONE',  ( 28.67810496033440515, -289.0500089654581757, -233.9239704021375701 ) ) ;
#11058=CARTESIAN_POINT ( 'NONE',  ( -112.4432852073904883, -272.7646693551740782, -253.3684160615795520 ) ) ;
#11059=CARTESIAN_POINT ( 'NONE',  ( -108.5787140985212318, -292.8215292307491495, -248.0214957618943004 ) ) ;
#11061=CARTESIAN_POINT ( 'NONE',  ( -55.63300648810263738, -294.3376638359845288, -190.3683826091709363 ) ) ;
#11063=CARTESIAN_POINT ( 'NONE',  ( -4.811872070706630922, -274.6246261199796095, -338.1383761130663856 ) ) ;
#11065=CARTESIAN_POINT ( 'NONE',  ( -71.73141684349430136, -293.8988845066755289, -338.3595576862630878 ) ) ;
#11066=CARTESIAN_POINT ( 'NONE',  ( -11.44636086817499177, -273.7470456629229147, -201.9452788165103243 ) ) ;
#11068=CARTESIAN_POINT ( 'NONE',  ( -37.24788492967900311, -290.5710802136277948, -344.0543941582762386 ) ) ;
#11069=B_SPLINE_SURFACE_WITH_KNOTS ( 'NONE', 3, 3, ( 
 ( #74222, #59101, #45318, #29293, #65770, #81781, #8879, #30677, #66664, #36854, #9341, #72833, #73315, #65299, #15075, #87481, #37758, #7501, #43936, #38226, #59577, #31156, #7959, #879, #22630, #60042, #1328, #29759, #67139, #2273, #43488, #22182, #51503, #24028, #73767, #79938, #8427, #52903, #405, #72384 ),
 ( #87942, #51050, #23577, #58188, #66212, #58639, #87030, #23093, #88879, #80391, #15535, #44864, #37306, #51976, #16012, #52444, #81318, #75166, #76568, #11691, #76097, #10748, #33462, #46262, #11230, #69001, #89818, #3666, #25428, #53374, #91208, #60502, #10279, #24979, #62365, #53853, #61894, #39605, #90727, #40542 ),
 ( #39149, #17870, #26376, #68060, #69457, #82718, #83646, #89338, #4132, #54306, #55264, #68529, #32554, #16931, #4588, #45792, #3186, #74703, #33003, #24493, #9824, #25887, #32070, #60967, #40084, #38697, #67604, #2732, #83180, #31612, #61446, #54769, #18329, #82260, #46722, #75625, #18810, #47667, #90277, #47185 ),
 ( #63790, #21135, #48127, #92154, #50004, #28256, #56684, #93555, #84580, #78898, #71342, #71821, #48598, #19729, #34416, #6941, #41960, #55728, #14045, #42908, #28713, #62855, #63323, #64728, #20678, #26840, #20207, #84119, #77030, #19269, #6472, #6004, #34878, #91688, #78444, #12160, #13124, #77498, #41004, #70873 ),
 ( #64272, #27791, #92620, #12645, #69927, #41490, #85056, #5546, #85531, #70420, #27310, #56197, #49549, #35350, #57144, #49085, #5069, #13580, #77983, #42431, #93101, #35814, #85985, #33951, #88313, #44295, #59461, #43376, #79830, #37204, #29175, #14970, #50947, #58534, #9232, #22077, #16360, #65656, #30563, #7390 ),
 ( #7848, #21601, #58071, #87379, #66560, #769, #22988, #15428, #36735, #51862, #38112, #23470, #22526, #43826, #66112, #1225, #51398, #52336, #15906, #72271, #50482, #36271, #73203, #65191, #295, #79383, #8322, #80288, #81214, #30107, #44763, #14521, #58989, #45211, #86924, #29654, #74113, #1681, #87837, #67022 ),
 ( #80755, #72726, #73663, #2158, #8774, #37652, #57598, #86442, #61785, #67497, #89700, #89233, #24866, #75982, #60857, #24385, #75062, #68420, #82146, #16821, #45679, #53749, #88776, #3550, #59937, #11110, #32439, #82615, #2628, #23924, #38594, #31963, #46158, #75517, #9714, #10173, #53264, #61338, #18225, #68892 ),
 ( #39043, #17762, #39498, #31507, #11582, #74586, #17302, #67954, #47556, #3079, #39977, #46616, #4022, #90617, #10639, #32897, #90175, #25323, #83534, #25779, #54660, #54203, #83071, #60395, #52794, #47075, #81673, #18693, #76461, #40430, #69348, #31047, #56088, #77390, #92510, #78794, #64161, #34309, #84472, #13019 ),
 ( #92994, #56575, #84014, #91087, #19162, #84941, #12052, #40899, #62252, #48973, #92047, #35236, #20092, #85428, #26258, #77870, #28152, #55152, #12527, #57041, #42325, #70768, #13938, #42796, #63686, #20576, #27677, #91580, #6364, #33839, #5442, #48019, #69818, #48490, #49448, #76924, #4953, #85879, #78336, #21031 ),
 ( #5901, #49899, #4478, #41377, #62748, #41855, #70311, #63215, #26736, #33355, #34771, #27201, #13478, #71236, #55623, #19622, #72621, #29546, #72170, #35713, #21971, #64627, #7286, #7743, #80638, #79727, #37095, #58426, #50844, #66004, #53507, #37541, #36626, #57958, #80182, #15320, #65547, #66452, #29997, #57497 ),
 ( #58882, #44180, #28608, #86813, #86340, #1116, #87728, #93453, #22418, #44653, #662, #17533, #71712, #87272, #36164, #8663, #22880, #31732, #65085, #43723, #73086, #29067, #51290, #15794, #8217, #51746, #21491, #73554, #2851, #14415, #60623, #185, #89461, #24622, #6839, #79274, #50370, #82384, #43272, #14869 ),
 ( #54898, #83299, #18447, #39267, #12287, #83775, #69120, #47305, #54428, #75283, #11351, #91337, #76220, #39730, #90391, #18931, #3789, #32195, #61100, #40204, #10402, #47786, #68184, #26499, #76687, #4246, #17989, #3305, #53969, #33126, #61558, #90850, #25095, #25547, #10867, #11812, #33589, #84241, #62015, #89940 ),
 ( #40663, #82836, #26966, #46841, #68653, #26012, #62981, #69583, #55390, #4711, #19391, #41131, #32672, #48254, #62498, #77156, #5205, #70064, #75744, #34079, #91814, #55857, #84710, #46383, #49671, #78106, #79510, #14647, #79032, #13705, #36403, #20340, #14186, #71950, #92755, #6606, #28379, #56328, #424, #63449 ),
 ( #50620, #35484, #21744, #5665, #42083, #93226, #85192, #70999, #13247, #20801, #65317, #6131, #72400, #27923, #86575, #92280, #7070, #57270, #58205, #71474, #64400, #19857, #43504, #48728, #49210, #7518, #35941, #27436, #77630, #64859, #35002, #63918, #43047, #29311, #70543, #12780, #86114, #34541, #21263, #93686 ),
 ( #56811, #41622, #50133, #42557, #85653, #28844, #57728, #78567, #22525, #73662, #6940, #50946, #8773, #80754, #15427, #52335, #81213, #8321, #30106, #66111, #36270, #44762, #72270, #43825, #64727, #14520, #86923, #37203, #35813, #43375, #37651, #58988, #30562, #7389, #65190, #22076, #59460, #768, #294, #66559 ),
 ( #21600, #79829, #23469, #73202, #79382, #72725, #42907, #93554, #71820, #87836, #58533, #87378, #50481, #1224, #28712, #65655, #29174, #57597, #29653, #88312, #58070, #86441, #51397, #14969, #1680, #7847, #36734, #80287, #44294, #22987, #51861, #15905, #46157, #90616, #9231, #54659, #3549, #31962, #60856, #23923 ),
 ( #2157, #31046, #75061, #74112, #82614, #45210, #90174, #53748, #39042, #81672, #38111, #52793, #17301, #31506, #89699, #88775, #60394, #74585, #46615, #32438, #54202, #24384, #67021, #24865, #16820, #68419, #45678, #47074, #9713, #83070, #75981, #3078, #18224, #59936, #38593, #17761, #67496, #2627, #89232, #10172 ),
 ( #11109, #39976, #67953, #75516, #53263, #82145, #10638, #39497, #61337, #25322, #68891, #4021, #32896, #61784, #25778, #16359, #64160, #49447, #19621, #69817, #92046, #27200, #77389, #78335, #41854, #69347, #76460, #4477, #41376, #91086, #26257, #47555, #34308, #12526, #20575, #5441, #70767, #11581, #63214, #13477 ),
 ( #48018, #42324, #5900, #71235, #19161, #55622, #56087, #40898, #48489, #92509, #84940, #20091, #40429, #34770, #6363, #55151, #70310, #76923, #63685, #48972, #18692, #84013, #33354, #77869, #35235, #92993, #28151, #62251, #33838, #83533, #13018, #12051, #27676, #4952, #62747, #91579, #56574, #85427, #26735, #84471 ),
 ( #42795, #71711, #86812, #21030, #29545, #85878, #37094, #661, #79726, #28607, #49898, #64626, #57957, #72169, #7742, #35712, #7285, #21490, #87271, #44179, #1115, #65084, #78793, #36625, #57496, #15319, #86339, #87727, #50369, #29996, #22879, #43722, #58881, #6838, #79273, #65546, #14414, #43271, #36163, #21970 ),
 ( #51745, #80637, #50843, #14868, #184, #13937, #29066, #93452, #72620, #58425, #66003, #22417, #51289, #80181, #73085, #8216, #37540, #15793, #44652, #73553, #8662, #66451, #1569, #57040, #82503, #16249, #23356, #45099, #82024, #37995, #66903, #88196, #74950, #24269, #61222, #46045, #17651, #52223, #10060, #90056 ),
 ( #25209, #68303, #2964, #39853, #68776, #89580, #46502, #53633, #23812, #32319, #59822, #31391, #81106, #2042, #74460, #24750, #74001, #30932, #54082, #75405, #18106, #88663, #52675, #9592, #46959, #17181, #81556, #10519, #16704, #45559, #39388, #75861, #9118, #30452, #67839, #38480, #38930, #3424, #31850, #67384 ),
 ( #82952, #10984, #2514, #60739, #59345, #89118, #60281, #53144, #4827, #62135, #34651, #19967, #56445, #33239, #69698, #70189, #55026, #33710, #12898, #48369, #41248, #54544, #84818, #63564, #40318, #62622, #90966, #48841, #5323, #32782, #11467, #25662, #34191, #85307, #42198, #76805, #69233, #12401, #40779, #91462 ),
 ( #78218, #63095, #4362, #26613, #13357, #90502, #3905, #77746, #19502, #77272, #26131, #91923, #61670, #55504, #83896, #83412, #84353, #49324, #19047, #18565, #27078, #47431, #47903, #11931, #55964, #41736, #70649, #92391, #27551, #5777, #20456, #76341, #72849, #37776, #30695, #51520, #59118, #80882, #15092, #52921 ),
 ( #16482, #9359, #87959, #74239, #56924, #895, #51995, #43952, #29778, #65786, #73332, #24046, #36871, #31173, #80407, #45338, #22198, #59595, #16030, #16947, #30227, #23112, #71111, #38243, #6242, #7977, #2290, #88445, #51067, #35111, #23594, #92872, #44881, #67157, #64031, #15554, #60059, #88897, #73783, #81800 ) ),
 .UNSPECIFIED., .F., .F., .F.,
 ( 4, 3, 3, 3, 3, 3, 3, 3, 4 ),
 ( 4, 3, 3, 3, 3, 3, 3, 3, 3, 3, 3, 3, 3, 4 ),
 ( 0.4999999999999952816, 0.5624999999999958922, 0.6249999999999964473, 0.6874999999999971134, 0.7499999999999976685, 0.8124999999999982236, 0.8749999999999988898, 0.9374999999999994449, 1.000000000000000000 ),
 ( -3.628684052071867067E-13, 0.06249999999944978735, 0.1249999999992624372, 0.1874999999990751010, 0.2499999999988877508, 0.3749999999985130783, 0.4999999999981383780, 0.6249999999977636778, 0.6874999999975763831, 0.7499999999973889775, 0.8124999999972015718, 0.8749999999970142772, 0.9374999999968269826, 0.9999999999966395769 ),
 .UNSPECIFIED. ) ;
#11070=CARTESIAN_POINT ( 'NONE',  ( -4.355686057685435486, -284.3713770222227026, -336.6174149818518231 ) ) ;
#11071=CARTESIAN_POINT ( 'NONE',  ( -111.3467839346178465, -291.7369300115220767, -289.4358684843848550 ) ) ;
#11072=CARTESIAN_POINT ( 'NONE',  ( -33.58046804292548160, -293.4137363237697400, -193.9467776616444326 ) ) ;
#11073=CARTESIAN_POINT ( 'NONE',  ( 18.83173772143145897, -294.0467148364512582, -316.9824101643395693 ) ) ;
#11074=CARTESIAN_POINT ( 'NONE',  ( -82.70804606998876807, -287.4321626089407005, -210.6376276157305654 ) ) ;
#11075=CARTESIAN_POINT ( 'NONE',  ( 21.61138255414765297, -282.3857777287969384, -319.8942790647038805 ) ) ;
#11076=CARTESIAN_POINT ( 'NONE',  ( -73.93090063162645720, -293.6136506036418155, -336.5298171532111269 ) ) ;
#11077=CARTESIAN_POINT ( 'NONE',  ( -21.72806210196183230, -282.6906465273069102, -345.7614781413406604 ) ) ;
#11079=CARTESIAN_POINT ( 'NONE',  ( 35.43180877955224872, -277.3171048313345750, -253.6949273144960557 ) ) ;
#11081=CARTESIAN_POINT ( 'NONE',  ( 30.89617123739170168, -295.8376638359844719, -254.7536222014695397 ) ) ;
#11082=CARTESIAN_POINT ( 'NONE',  ( -90.47988972230045590, -275.9340790327501622, -324.4405203246855081 ) ) ;
#11084=CARTESIAN_POINT ( 'NONE',  ( -24.06045461068103108, -282.3855664621608526, -342.2053728606200025 ) ) ;
#11086=CARTESIAN_POINT ( 'NONE',  ( -109.2388601609837480, -280.0947830713159874, -243.7729323447709362 ) ) ;
#11087=CARTESIAN_POINT ( 'NONE',  ( 20.11862170518067217, -285.9185702876018240, -219.3794757253718331 ) ) ;
#11088=CARTESIAN_POINT ( 'NONE',  ( -3.188310742052926194, -294.2699080036458668, -204.6989522474358125 ) ) ;
#11089=CARTESIAN_POINT ( 'NONE',  ( 33.96587379092136416, -276.8088303427197729, -243.4971957844319093 ) ) ;
#11090=CARTESIAN_POINT ( 'NONE',  ( 35.59756893262619570, -277.1594066246558441, -293.4514038526494915 ) ) ;
#11091=CARTESIAN_POINT ( 'NONE',  ( -68.03935441109793203, -277.3000987560183717, -336.6066861282340028 ) ) ;
#11092=CARTESIAN_POINT ( 'NONE',  ( -70.08206762311330351, -299.6199537713510495, -203.0699835924160084 ) ) ;
#11093=CARTESIAN_POINT ( 'NONE',  ( -108.2618046777853209, -282.8633569964112553, -246.3166656167947792 ) ) ;
#11094=CARTESIAN_POINT ( 'NONE',  ( 17.47753067357390577, -292.4757889552715824, -216.2435132604818193 ) ) ;
#11095=CARTESIAN_POINT ( 'NONE',  ( 37.04844308345818149, -289.3616629136205347, -286.9297551506215314 ) ) ;
#11097=CARTESIAN_POINT ( 'NONE',  ( 35.73145807775177474, -292.5496759711669483, -276.2381599965387977 ) ) ;
#11099=CARTESIAN_POINT ( 'NONE',  ( -76.84894947634538198, -290.1091620702991918, -204.8953367990457650 ) ) ;
#11100=CARTESIAN_POINT ( 'NONE',  ( 24.86810874138845406, -292.6908015312446878, -232.0286543885544290 ) ) ;
#11102=CARTESIAN_POINT ( 'NONE',  ( -54.41934902124399542, -290.3461143080086799, -345.1808836089857095 ) ) ;
#11103=CARTESIAN_POINT ( 'NONE',  ( -108.9888072818816482, -279.3955602562056129, -255.7866873382242829 ) ) ;
#11104=CARTESIAN_POINT ( 'NONE',  ( -101.2843389529055713, -296.0319792565589978, -227.9953709198669287 ) ) ;
#11105=CARTESIAN_POINT ( 'NONE',  ( -4.824601086436063113, -287.1206635216473728, -200.6764635957316329 ) ) ;
#11106=CARTESIAN_POINT ( 'NONE',  ( 16.28141815142114979, -287.1219776718527328, -215.1315473029715122 ) ) ;
#11107=CARTESIAN_POINT ( 'NONE',  ( -101.7878928193862151, -284.4164033898601929, -304.8020270895105455 ) ) ;
#11108=CARTESIAN_POINT ( 'NONE',  ( 25.10643563140649448, -22.76097397130827815, -345.0702719944544583 ) ) ;
#11109=CARTESIAN_POINT ( 'NONE',  ( 201.5605228849236426, 295.4036489450776344, -54.00000000002459188 ) ) ;
#11110=CARTESIAN_POINT ( 'NONE',  ( -47.88318689526796845, -154.9995436933450605, -361.3103295439817089 ) ) ;
#11111=CARTESIAN_POINT ( 'NONE',  ( 20.81610211598217930, -274.1262451277162882, -225.9527498682777775 ) ) ;
#11112=CARTESIAN_POINT ( 'NONE',  ( 11.94540050142956567, -275.2684591037336190, -324.6979152150947243 ) ) ;
#11113=CARTESIAN_POINT ( 'NONE',  ( -112.5390163706340729, -296.2642382456113523, -254.0241914527857148 ) ) ;
#11114=CARTESIAN_POINT ( 'NONE',  ( 185.8120907569735891, 260.3495500449395195, -151.3467373205649835 ) ) ;
#11115=CARTESIAN_POINT ( 'NONE',  ( 38.88771076079248701, -274.3189168564398983, -276.8707406564970483 ) ) ;
#11116=CARTESIAN_POINT ( 'NONE',  ( -57.15413860319132766, -275.5533179835579176, -198.9953851041864823 ) ) ;
#11118=CARTESIAN_POINT ( 'NONE',  ( -31.94217931762041118, -299.0594502518147237, -193.5955712977170151 ) ) ;
#11119=CARTESIAN_POINT ( 'NONE',  ( -66.34769653104673637, -289.9346832550450586, -337.4721724312433935 ) ) ;
#11120=CARTESIAN_POINT ( 'NONE',  ( -111.8096161828856339, -297.1168942843181640, -289.3532753395764416 ) ) ;
#11121=CARTESIAN_POINT ( 'NONE',  ( -112.2444462341738642, -296.8237278202183802, -287.9994803679311985 ) ) ;
#11122=CARTESIAN_POINT ( 'NONE',  ( -58.40620969087483161, -295.4988571916826459, -340.2559421211702215 ) ) ;
#11124=AXIS2_PLACEMENT_3D ( 'NONE', #91135, #39538, #68459 ) ;
#11125=CARTESIAN_POINT ( 'NONE',  ( -69.66243976247527314, -279.3943817688218019, -338.6737756042700767 ) ) ;
#11127=CARTESIAN_POINT ( 'NONE',  ( -14.24025656469665080, -279.8514351758454382, -196.9169089891026374 ) ) ;
#11129=CARTESIAN_POINT ( 'NONE',  ( -16.30184157120112332, -277.7148091657475106, -340.5622356392174765 ) ) ;
#11130=CARTESIAN_POINT ( 'NONE',  ( 26.80558192295882947, -277.8543387554825586, -311.1910231098851227 ) ) ;
#11131=CARTESIAN_POINT ( 'NONE',  ( -39.93221443359873746, -275.1046283449192629, -345.6845682911584845 ) ) ;
#11132=CARTESIAN_POINT ( 'NONE',  ( -36.74185794118342585, -274.5522376084319944, -197.2896163155269846 ) ) ;
#11133=CARTESIAN_POINT ( 'NONE',  ( -58.05337773407750745, -296.3539720910771393, -199.7466624756449391 ) ) ;
#11135=CARTESIAN_POINT ( 'NONE',  ( -85.10363866667154298, -277.8996709114925920, -325.6349349247532814 ) ) ;
#11137=CARTESIAN_POINT ( 'NONE',  ( -52.52374249793685834, -274.6654095900231027, -194.9830589272008012 ) ) ;
#11138=CARTESIAN_POINT ( 'NONE',  ( 25.43738772882143095, -286.8196198140358320, -314.1794402345108210 ) ) ;
#11139=CARTESIAN_POINT ( 'NONE',  ( -27.29044299662773199, -276.1799215197347621, -195.9856428099257926 ) ) ;
#11142=CARTESIAN_POINT ( 'NONE',  ( -56.11687207286747991, -288.4972695515995724, -341.1251405500296983 ) ) ;
#11144=CARTESIAN_POINT ( 'NONE',  ( -112.8965053268430694, -284.0833714990520775, -255.7739410976076044 ) ) ;
#11145=CARTESIAN_POINT ( 'NONE',  ( 36.70165498353557609, -279.7688454439426096, -268.5812678106142357 ) ) ;
#11146=CARTESIAN_POINT ( 'NONE',  ( 28.31524924824635647, -279.6779163578821681, -237.0134559978289133 ) ) ;
#11147=CARTESIAN_POINT ( 'NONE',  ( -33.13326652609070777, -284.1852695871455126, -195.9893681649109567 ) ) ;
#11148=CARTESIAN_POINT ( 'NONE',  ( 34.14175854281398159, -289.8456935641403902, -293.0993790409129360 ) ) ;
#11149=CARTESIAN_POINT ( 'NONE',  ( -110.3627934562378385, -279.8609853202134445, -262.4534051004393405 ) ) ;
#11151=CARTESIAN_POINT ( 'NONE',  ( -47.49843290267460816, -293.9233500554501575, -195.9996247949634380 ) ) ;
#11153=CARTESIAN_POINT ( 'NONE',  ( -113.0323485360361246, -276.8841812740284922, -263.0883200953797996 ) ) ;
#11154=CARTESIAN_POINT ( 'NONE',  ( -61.81614764838461440, -278.0301026354008513, -339.2981228691048159 ) ) ;
#11155=CARTESIAN_POINT ( 'NONE',  ( -13.96727668575623404, -284.7497394021139030, -341.8010560670164182 ) ) ;
#11156=FACE_BOUND ( 'NONE', #90130, .T. ) ;
#11157=CARTESIAN_POINT ( 'NONE',  ( -56.89424512180426063, -291.2223974544353382, -343.4015707551772607 ) ) ;
#11158=CARTESIAN_POINT ( 'NONE',  ( -96.08379003318228229, -295.1929095770927347, -223.7107914564602993 ) ) ;
#11160=CARTESIAN_POINT ( 'NONE',  ( -2.287430849810337730, -285.7012486814879253, -201.9698130193444570 ) ) ;
#11161=CARTESIAN_POINT ( 'NONE',  ( -95.73502178914699812, -289.5805541775005167, -225.2317439257451213 ) ) ;
#11163=CARTESIAN_POINT ( 'NONE',  ( 25.79069818050878737, -274.7507879289541393, -307.9848307317479907 ) ) ;
#11164=CARTESIAN_POINT ( 'NONE',  ( 17.98560915142196137, -292.3882150695460496, -319.8752689016915269 ) ) ;
#11167=CARTESIAN_POINT ( 'NONE',  ( -27.91536765317002988, -290.6495020049017626, -194.5857227514489125 ) ) ;
#11168=CARTESIAN_POINT ( 'NONE',  ( -73.97020223445493059, -287.1571125274352312, -206.2778005892703845 ) ) ;
#11169=CARTESIAN_POINT ( 'NONE',  ( 0.1988940112167022212, -286.7996880825637618, -336.4862777388386803 ) ) ;
#11170=CARTESIAN_POINT ( 'NONE',  ( -62.78348526920450468, -287.1397898224032588, -201.2554080310264055 ) ) ;
#11172=CARTESIAN_POINT ( 'NONE',  ( -54.80477001058553554, -286.6248540998305998, -199.2619370136571604 ) ) ;
#11173=CARTESIAN_POINT ( 'NONE',  ( 36.46481204283844590, -295.7262723003140081, -285.5599852940453047 ) ) ;
#11174=CARTESIAN_POINT ( 'NONE',  ( -107.3319585571128414, -276.2635152955796229, -298.8335242858804008 ) ) ;
#11175=CARTESIAN_POINT ( 'NONE',  ( -114.3567419237675580, -278.9057259920187448, -268.7389283780404412 ) ) ;
#11177=CARTESIAN_POINT ( 'NONE',  ( -76.40349984469487765, -289.6143601046818503, -205.6208816450483141 ) ) ;
#11178=CARTESIAN_POINT ( 'NONE',  ( -107.5761041906091435, -278.1476022556817043, -302.0523627193825860 ) ) ;
#11179=CARTESIAN_POINT ( 'NONE',  ( 98.12082082284621265, -301.7359631804335436, -195.6703527335122601 ) ) ;
#11182=CARTESIAN_POINT ( 'NONE',  ( -104.2544786422812138, -276.2626393102725615, -302.6289431065487747 ) ) ;
#11183=CARTESIAN_POINT ( 'NONE',  ( 37.28529038273786966, -279.6543336527219026, -278.3319625602289875 ) ) ;
#11185=CARTESIAN_POINT ( 'NONE',  ( -9.483136583787503682, -275.1744817237452594, -341.4006013002754685 ) ) ;
#11186=CARTESIAN_POINT ( 'NONE',  ( -100.7532965277512318, -297.5600158377420712, -308.0072204082302960 ) ) ;
#11187=CARTESIAN_POINT ( 'NONE',  ( -13.53101158818511962, -281.6704036963191697, -343.2620344406865911 ) ) ;
#11188=CARTESIAN_POINT ( 'NONE',  ( -106.9341234464503714, -297.7970769889863618, -247.3901114819853149 ) ) ;
#11189=CARTESIAN_POINT ( 'NONE',  ( -97.85428625583519135, -298.4965165734280390, -223.5262396483698240 ) ) ;
#11190=CARTESIAN_POINT ( 'NONE',  ( -71.91399351379897098, -273.2488685131103239, -205.9864766387333930 ) ) ;
#11191=CARTESIAN_POINT ( 'NONE',  ( -1.505615463905816354, -294.5273562414528215, -204.4619727063512471 ) ) ;
#11192=CARTESIAN_POINT ( 'NONE',  ( 39.34763579612192075, -287.8052487256001655, -277.2709486604872495 ) ) ;
#11193=CARTESIAN_POINT ( 'NONE',  ( 34.02929029170060460, -274.0196506963127376, -295.9417315768594108 ) ) ;
#11194=CARTESIAN_POINT ( 'NONE',  ( -60.02930083976117714, -289.1716111294249458, -343.9428601366946623 ) ) ;
#11196=CARTESIAN_POINT ( 'NONE',  ( 34.98972816454642754, -286.7627752598561983, -281.9114786876830863 ) ) ;
#11197=CARTESIAN_POINT ( 'NONE',  ( -106.5125022705141475, -288.9305696947652677, -241.3714512539633859 ) ) ;
#11199=CARTESIAN_POINT ( 'NONE',  ( -104.9628119525177112, -256.0684274861638983, -326.9234398911233939 ) ) ;
#11201=CARTESIAN_POINT ( 'NONE',  ( 34.58116575261266235, -287.2291563452496916, -283.2098457517813017 ) ) ;
#11203=CARTESIAN_POINT ( 'NONE',  ( -112.1332027681788759, -285.7103376914195678, -253.0680168422167355 ) ) ;
#11204=CARTESIAN_POINT ( 'NONE',  ( 37.53447219344495522, -292.3979470227529305, -253.3794029679523021 ) ) ;
#11205=CARTESIAN_POINT ( 'NONE',  ( 20.44595780854720246, -282.4745828335325086, -220.6721084005253601 ) ) ;
#11206=CARTESIAN_POINT ( 'NONE',  ( 28.85147717333750350, -282.3651916689637460, -231.9975734320101708 ) ) ;
#11207=CARTESIAN_POINT ( 'NONE',  ( -16.13452854233381117, -282.6034857096240103, -340.2127885268016598 ) ) ;
#11208=CARTESIAN_POINT ( 'NONE',  ( 30.98655835208749210, -277.9579614454664807, -301.2844059510375132 ) ) ;
#11209=CARTESIAN_POINT ( 'NONE',  ( -112.8886848000154401, -296.7391954051330458, -255.4052924458295024 ) ) ;
#11211=CARTESIAN_POINT ( 'NONE',  ( -96.68945355043678092, -274.4712446624611175, -226.9280982618618623 ) ) ;
#11212=CARTESIAN_POINT ( 'NONE',  ( -111.8866982839125797, -288.6335967337550983, -265.6062723070377274 ) ) ;
#11213=CARTESIAN_POINT ( 'NONE',  ( -108.3201243057135343, -271.5948065558897611, -251.4796499309283035 ) ) ;
#11215=DIRECTION ( 'NONE',  ( 1.000000000000000000, 0.000000000000000000, 0.000000000000000000 ) ) ;
#11216=CARTESIAN_POINT ( 'NONE',  ( -111.3005844235002542, -286.3572657036031615, -279.2541925294103748 ) ) ;
#11218=( BOUNDED_CURVE ( )  B_SPLINE_CURVE ( 2, ( #17928, #39667, #68589, #83239, #33521, #56255, #70929, #19323, #12217, #18386, #84638, #12708, #48658, #18868, #27366, #54828, #26432, #47243, #90787, #69515, #19787, #83706, #91746, #54365, #5600, #62910, #48185, #25947, #76155, #33061, #55325, #40601, #69989, #4187, #4646, #47725, #55785, #41548, #34932, #20265, #5129, #84175, #76625, #77559, #34006, #11288, #91268, #34474, #26897, #11748, #70472, #61950, #42013, #62427, #63380, #41063, #92210, #77086, #69058, #78038, #85115, #49141, #13178, #6060, #63847, #25486, #40142, #14572, #92679, #57198, #346, #6996, #22127, #50995, #42486, #27849, #79880, #56738, #71399, #42969, #20731, #58586, #15020, #78497, #85584, #71874, #29703, #43428, #49601, #13635, #72323, #86499, #87425, #7444, #43880, #6532, #36326, #22573, #35408, #35868, #51447, #64328, #50059, #28768, #64785, #65240, #78955, #57651, #7901, #29233, #58128, #93154, #72776, #80336, #28309, #21662, #86039, #36790, #86973, #21188, #14105, #93610, #50538 ),
 .UNSPECIFIED., .F., .F. ) 
 B_SPLINE_CURVE_WITH_KNOTS ( ( 3, 2, 2, 2, 2, 2, 2, 2, 2, 2, 2, 2, 2, 2, 2, 2, 2, 2, 2, 2, 2, 2, 2, 2, 2, 2, 2, 2, 2, 2, 2, 2, 2, 2, 2, 2, 2, 2, 2, 2, 2, 2, 2, 2, 2, 2, 2, 2, 2, 2, 2, 2, 2, 2, 2, 2, 2, 2, 2, 2, 2, 3 ),
 ( -0.05135551144988959038, 0.000000000000000000, 0.01428571428571429047, 0.02857142857142856707, 0.04285714285714285754, 0.05714285714285713413, 0.07142857142857142461, 0.08571428571428571508, 0.1000000000000000056, 0.1142857142857142405, 0.1285714285714285587, 0.1428571428571428492, 0.1571428571428571397, 0.1714285714285714302, 0.1857142857142857206, 0.2000000000000000111, 0.2142857142857143016, 0.2285714285714285365, 0.2428571428571429380, 0.2571428571428571175, 0.2714285714285713524, 0.2857142857142856984, 0.2999999999999999889, 0.3142857142857142794, 0.3285714285714285698, 0.3428571428571428603, 0.3571428571428571508, 0.3714285714285714413, 0.3857142857142857317, 0.4000000000000000222, 0.4142857142857143127, 0.4285714285714285476, 0.4428571428571428381, 0.4571428571428570731, 0.4714285714285714191, 0.4857142857142857650, 0.5000000000000000000, 0.5142857142857142350, 0.5285714285714285809, 0.5428571428571428159, 0.5571428571428571619, 0.5714285714285713969, 0.5857142857142857428, 0.5999999999999999778, 0.6142857142857143238, 0.6285714285714285587, 0.6428571428571429047, 0.6571428571428571397, 0.6714285714285713746, 0.6857142857142857206, 0.6999999999999999556, 0.7142857142857143016, 0.7285714285714285365, 0.7428571428571428825, 0.7571428571428571175, 0.7714285714285714635, 0.7857142857142856984, 0.8000000000000000444, 0.8142857142857142794, 0.8285714285714287364, 0.8428571428571428603, 0.8500000000000000888 ),
 .UNSPECIFIED. ) 
 CURVE ( )  GEOMETRIC_REPRESENTATION_ITEM ( )  RATIONAL_B_SPLINE_CURVE ( ( 1.000000000000000000, 1.000000000000000000, 1.000000000000000000, 0.9749279121818236193, 1.000000000000000000, 0.9749279121818236193, 1.000000000000000000, 0.9749279121818236193, 1.000000000000000000, 0.9749279121818236193, 1.000000000000000000, 0.9749279121818236193, 1.000000000000000000, 0.9749279121818236193, 1.000000000000000000, 0.9749279121818236193, 1.000000000000000000, 0.9749279121818236193, 1.000000000000000000, 0.9749279121818236193, 1.000000000000000000, 0.9749279121818236193, 1.000000000000000000, 0.9749279121818236193, 1.000000000000000000, 0.9749279121818236193, 1.000000000000000000, 0.9749279121818236193, 1.000000000000000000, 0.9749279121818236193, 1.000000000000000000, 0.9749279121818236193, 1.000000000000000000, 0.9749279121818236193, 1.000000000000000000, 0.9749279121818236193, 1.000000000000000000, 0.9749279121818236193, 1.000000000000000000, 0.9749279121818236193, 1.000000000000000000, 0.9749279121818236193, 1.000000000000000000, 0.9749279121818236193, 1.000000000000000000, 0.9749279121818236193, 1.000000000000000000, 0.9749279121818236193, 1.000000000000000000, 0.9749279121818236193, 1.000000000000000000, 0.9749279121818236193, 1.000000000000000000, 0.9749279121818236193, 1.000000000000000000, 0.9749279121818236193, 1.000000000000000000, 0.9749279121818236193, 1.000000000000000000, 0.9749279121818236193, 1.000000000000000000, 0.9749279121818236193, 1.000000000000000000, 0.9749279121818236193, 1.000000000000000000, 0.9749279121818236193, 1.000000000000000000, 0.9749279121818236193, 1.000000000000000000, 0.9749279121818236193, 1.000000000000000000, 0.9749279121818236193, 1.000000000000000000, 0.9749279121818236193, 1.000000000000000000, 0.9749279121818236193, 1.000000000000000000, 0.9749279121818236193, 1.000000000000000000, 0.9749279121818236193, 1.000000000000000000, 0.9749279121818236193, 1.000000000000000000, 0.9749279121818236193, 1.000000000000000000, 0.9749279121818236193, 1.000000000000000000, 0.9749279121818236193, 1.000000000000000000, 0.9749279121818236193, 1.000000000000000000, 0.9749279121818236193, 1.000000000000000000, 0.9749279121818236193, 1.000000000000000000, 0.9749279121818236193, 1.000000000000000000, 0.9749279121818236193, 1.000000000000000000, 0.9749279121818236193, 1.000000000000000000, 0.9749279121818236193, 1.000000000000000000, 0.9749279121818236193, 1.000000000000000000, 0.9749279121818236193, 1.000000000000000000, 0.9749279121818236193, 1.000000000000000000, 0.9749279121818236193, 1.000000000000000000, 0.9749279121818236193, 1.000000000000000000, 0.9749279121818236193, 1.000000000000000000, 0.9749279121818236193, 1.000000000000000000, 0.9749279121818236193, 1.000000000000000000, 0.9749279121818236193, 1.000000000000000000, 0.9874639560909115321, 0.9874639560909117542 ) ) 
 REPRESENTATION_ITEM ( '' )  );
#11219=CARTESIAN_POINT ( 'NONE',  ( 1.624269386226377510, -295.6235624648946896, -336.4152301141319867 ) ) ;
#11221=CARTESIAN_POINT ( 'NONE',  ( -95.99858010412029330, -284.5924704743349594, -313.9875216841513179 ) ) ;
#11222=CARTESIAN_POINT ( 'NONE',  ( 12.54259940834403686, -275.4351481904558909, -328.7081562284523670 ) ) ;
#11223=CARTESIAN_POINT ( 'NONE',  ( -58.91804095993250456, -292.4315309027696230, -196.5520785455045996 ) ) ;
#11224=CARTESIAN_POINT ( 'NONE',  ( -105.5565534029861539, -283.1216778404532306, -237.3908393902971170 ) ) ;
#11225=CARTESIAN_POINT ( 'NONE',  ( -56.18771979708773046, -292.1492153310924778, -195.6699206426692399 ) ) ;
#11226=CARTESIAN_POINT ( 'NONE',  ( -110.3272207071332929, -290.8385778176651684, -273.9142166232599038 ) ) ;
#11230=CARTESIAN_POINT ( 'NONE',  ( -38.49763412114499062, -140.3826428618228590, -361.0438956898904621 ) ) ;
#11231=CARTESIAN_POINT ( 'NONE',  ( -112.9099497434466457, -285.9339238109115513, -281.3236272611336517 ) ) ;
#11232=CARTESIAN_POINT ( 'NONE',  ( -54.49178911615187104, -292.7666405000204009, -345.3538533559490702 ) ) ;
#11234=CARTESIAN_POINT ( 'NONE',  ( -3.490821103498019884, -281.5146541893625454, -335.4008997861424746 ) ) ;
#11235=CARTESIAN_POINT ( 'NONE',  ( 24.34816871883806755, -275.8315699416610300, -316.4057091225723184 ) ) ;
#11236=CARTESIAN_POINT ( 'NONE',  ( -108.1884511879738824, -280.8665737776762512, -246.1027318723067765 ) ) ;
#11237=CARTESIAN_POINT ( 'NONE',  ( 181.6399435233035149, 251.7122595193576728, -165.5316943122344071 ) ) ;
#11238=CARTESIAN_POINT ( 'NONE',  ( -81.23801407186208223, -282.2103034980410712, -332.9692416852994370 ) ) ;
#11239=CARTESIAN_POINT ( 'NONE',  ( -109.6935897988081621, -282.3352877322018344, -288.7200631314100860 ) ) ;
#11240=CARTESIAN_POINT ( 'NONE',  ( 52.07892576469384949, -300.9172225385302113, -194.3480566079236382 ) ) ;
#11242=CARTESIAN_POINT ( 'NONE',  ( -50.47612140227846567, -295.7167720108961362, -342.2323599314181592 ) ) ;
#11244=CARTESIAN_POINT ( 'NONE',  ( 35.39821468066580934, -292.0994536180252794, -259.8659633004283478 ) ) ;
#11245=CARTESIAN_POINT ( 'NONE',  ( 38.63635908846916323, -276.3562667224822462, -282.5550258268467587 ) ) ;
#11246=CARTESIAN_POINT ( 'NONE',  ( -31.33971031512739103, -274.1300316492268507, -197.5956257076479119 ) ) ;
#11247=CARTESIAN_POINT ( 'NONE',  ( 11.59904624462071432, -273.6330006578010625, -211.2472377990444556 ) ) ;
#11249=CARTESIAN_POINT ( 'NONE',  ( -5.483631870131095987, -272.4710459953950590, -202.4497445252075067 ) ) ;
#11252=CARTESIAN_POINT ( 'NONE',  ( 22.07049152028501382, -283.2303133990907327, -313.3292992823072609 ) ) ;
#11253=CARTESIAN_POINT ( 'NONE',  ( 30.18700024344522248, -283.7673574052660683, -305.2014485994206439 ) ) ;
#11254=CARTESIAN_POINT ( 'NONE',  ( -104.6882332572437235, -284.2833620694008800, -241.7997736497220842 ) ) ;
#11255=CARTESIAN_POINT ( 'NONE',  ( -76.80059102335336263, -275.9895532070642616, -332.7865749132354836 ) ) ;
#11256=CARTESIAN_POINT ( 'NONE',  ( -43.00388115797979083, -284.9846585319517658, -344.4310038557687221 ) ) ;
#11257=CARTESIAN_POINT ( 'NONE',  ( -85.57350775601103976, -276.2131403585453882, -326.1458772527687984 ) ) ;
#11259=CARTESIAN_POINT ( 'NONE',  ( -19.20840370434564548, -275.3705625465728986, -199.2774243313589579 ) ) ;
#11262=CARTESIAN_POINT ( 'NONE',  ( -113.8840200522656971, -279.4467421975192565, -263.0395027813385127 ) ) ;
#11266=CARTESIAN_POINT ( 'NONE',  ( -112.3726856812481856, -286.2741628816356751, -281.2502084701395120 ) ) ;
#11267=CARTESIAN_POINT ( 'NONE',  ( -0.6858837335020224746, -293.7493308390761513, -333.7352271971253117 ) ) ;
#11268=CARTESIAN_POINT ( 'NONE',  ( -102.2197270515946883, -289.3578092508161603, -311.7405282011702070 ) ) ;
#11269=CARTESIAN_POINT ( 'NONE',  ( 34.99636457891098473, -285.9964633386975947, -286.0786469452647793 ) ) ;
#11270=CARTESIAN_POINT ( 'NONE',  ( -42.69905825203463934, -284.5579945653087748, -196.9544286588893556 ) ) ;
#11271=CARTESIAN_POINT ( 'NONE',  ( -63.13313071697616863, -289.9514142737637030, -200.9869432382342609 ) ) ;
#11272=CARTESIAN_POINT ( 'NONE',  ( -64.18638933987271855, -284.6154590157877919, -338.6728531838838308 ) ) ;
#11273=CARTESIAN_POINT ( 'NONE',  ( 37.32873527455178930, -273.4550046209459424, -262.8077666946611544 ) ) ;
#11274=CARTESIAN_POINT ( 'NONE',  ( 24.07073671188498309, -285.3465645313724508, -225.2506644459180052 ) ) ;
#11275=CARTESIAN_POINT ( 'NONE',  ( -35.55779474766005421, -300.0746396841030901, -195.3605010756353408 ) ) ;
#11276=CARTESIAN_POINT ( 'NONE',  ( 24.33251116992141760, -286.1347439301002282, -313.4192726471200672 ) ) ;
#11277=CARTESIAN_POINT ( 'NONE',  ( -35.66940553494461597, -281.0148643754564546, -197.1324754626337210 ) ) ;
#11278=CARTESIAN_POINT ( 'NONE',  ( -84.00610051449423565, -291.6913500165445043, -329.3551105709826174 ) ) ;
#11281=CARTESIAN_POINT ( 'NONE',  ( -52.96712810417530903, -297.1709372653128298, -344.3413590588211832 ) ) ;
#11282=CARTESIAN_POINT ( 'NONE',  ( -13.65368674449415920, -278.3593261084973278, -199.1452728415090974 ) ) ;
#11283=CARTESIAN_POINT ( 'NONE',  ( -68.25440222016531777, -290.8535520384341453, -200.0007541048808264 ) ) ;
#11284=CARTESIAN_POINT ( 'NONE',  ( -97.85085635573823026, -294.3693145329717140, -312.6113538220226928 ) ) ;
#11285=CARTESIAN_POINT ( 'NONE',  ( 34.24452696001080199, -280.0190287886448459, -253.7281515909492384 ) ) ;
#11286=CARTESIAN_POINT ( 'NONE',  ( -3.427220608014195591, -272.5832734608253531, -204.0812626408091148 ) ) ;
#11287=CARTESIAN_POINT ( 'NONE',  ( 36.13569879432272103, -294.9083761019044232, -273.4933972702096980 ) ) ;
#11288=CARTESIAN_POINT ( 'NONE',  ( -20.19161114001083490, -291.3376638359845288, -345.3538533559490702 ) ) ;
#11289=CARTESIAN_POINT ( 'NONE',  ( -101.0600855105126072, -294.4739017096634939, -312.4409384456258181 ) ) ;
#11290=CARTESIAN_POINT ( 'NONE',  ( 38.22679833462696308, -291.8990209280674435, -278.8048312412259406 ) ) ;
#11292=CARTESIAN_POINT ( 'NONE',  ( -38.92833475056011849, -293.4571351699126467, -196.7889934427387857 ) ) ;
#11294=CARTESIAN_POINT ( 'NONE',  ( 30.73957360934411653, -294.7140600771061827, -297.2867503812493624 ) ) ;
#11296=CARTESIAN_POINT ( 'NONE',  ( -4.895389037928816300, -280.6471767272557258, -338.3873798393946117 ) ) ;
#11297=CARTESIAN_POINT ( 'NONE',  ( 10.29152059668689922, -294.3730051613461001, -325.6790742299260728 ) ) ;
#11298=CARTESIAN_POINT ( 'NONE',  ( 15.75353287994514240, -282.3249805648094366, -326.1275615828414516 ) ) ;
#11299=CARTESIAN_POINT ( 'NONE',  ( -69.18158589412249171, -283.1263464489459807, -340.4609476158051962 ) ) ;
#11300=CARTESIAN_POINT ( 'NONE',  ( -81.50960561043548580, -287.6540168513712388, -330.8344276423498513 ) ) ;
#11302=CARTESIAN_POINT ( 'NONE',  ( 21.97200015200688838, -280.6818441227378003, -318.3879005566156479 ) ) ;
#11304=CARTESIAN_POINT ( 'NONE',  ( -31.86264499555948504, -287.9050084939606222, -346.9083810122533578 ) ) ;
#11306=CARTESIAN_POINT ( 'NONE',  ( -38.33281831385887983, -296.6649102561964355, -344.1544652583818333 ) ) ;
#11307=CARTESIAN_POINT ( 'NONE',  ( -1.726156742267933364, -278.0148366805206024, -337.9639238675458728 ) ) ;
#11308=CARTESIAN_POINT ( 'NONE',  ( -109.6421324285941807, -278.3584588987321808, -259.7764014511412825 ) ) ;
#11309=CARTESIAN_POINT ( 'NONE',  ( 35.45191640392692989, -293.4006018236302680, -245.0981516801702469 ) ) ;
#11311=CARTESIAN_POINT ( 'NONE',  ( -11.22317909835527239, -280.7944196730981048, -341.3190038640871080 ) ) ;
#11312=CARTESIAN_POINT ( 'NONE',  ( -7.162368059646126994, -291.5168249590747109, -203.6331900611855019 ) ) ;
#11313=CARTESIAN_POINT ( 'NONE',  ( -112.3093488958750612, -294.5976597207110217, -266.8040562119289802 ) ) ;
#11316=CARTESIAN_POINT ( 'NONE',  ( -20.84036663345083085, -294.3423741473930022, -341.5869574905818808 ) ) ;
#11318=CARTESIAN_POINT ( 'NONE',  ( 34.45848030099739390, -291.0523547857347353, -270.3937649182068412 ) ) ;
#11319=CARTESIAN_POINT ( 'NONE',  ( -9.205420001057850854, -297.4550882046272022, -193.6007765762892916 ) ) ;
#11320=CARTESIAN_POINT ( 'NONE',  ( 35.28768738530330040, -279.9688531837792311, -292.1117000145759448 ) ) ;
#11321=CARTESIAN_POINT ( 'NONE',  ( 0.02818890718441586715, -287.8538985787386650, -203.5869766456557386 ) ) ;
#11322=CARTESIAN_POINT ( 'NONE',  ( 5.842915620406163413, -288.2818276730639013, -329.2806252334829651 ) ) ;
#11323=CARTESIAN_POINT ( 'NONE',  ( -79.00821737978208148, -279.1450924438626657, -331.2065406280355546 ) ) ;
#11324=CARTESIAN_POINT ( 'NONE',  ( -37.85168605816453891, -299.8058200165792186, -196.3495382743187179 ) ) ;
#11325=CARTESIAN_POINT ( 'NONE',  ( -108.5610877620571983, -277.1135405807749521, -288.1592224866163860 ) ) ;
#11327=CARTESIAN_POINT ( 'NONE',  ( -110.1011692115127261, -272.7031827280777065, -245.1607278428051586 ) ) ;
#11328=CARTESIAN_POINT ( 'NONE',  ( -110.8370009187345602, -292.3183412605241074, -282.2629316736753253 ) ) ;
#11329=CARTESIAN_POINT ( 'NONE',  ( 10.70979577105156011, -296.0011728215579296, -329.5687454362955577 ) ) ;
#11331=CARTESIAN_POINT ( 'NONE',  ( -90.66143039088635192, -290.4842294239578564, -320.4440202816364831 ) ) ;
#11333=CARTESIAN_POINT ( 'NONE',  ( -110.7000583586131199, -296.9128819636652565, -293.4673548077265082 ) ) ;
#11334=CARTESIAN_POINT ( 'NONE',  ( -83.49484891535782083, -289.5669206786536733, -210.2101347911883806 ) ) ;
#11335=CARTESIAN_POINT ( 'NONE',  ( -93.65018486062362513, -297.6018534989476620, -217.7943255906305922 ) ) ;
#11338=CARTESIAN_POINT ( 'NONE',  ( -101.1152550013760276, -292.6291387553094410, -228.3658891274201892 ) ) ;
#11339=CARTESIAN_POINT ( 'NONE',  ( 13.79469577742117714, -295.1948066931273615, -206.1857440867352693 ) ) ;
#11340=CARTESIAN_POINT ( 'NONE',  ( -108.7272761255729847, -286.2619989184202041, -292.8139121584833902 ) ) ;
#11341=CARTESIAN_POINT ( 'NONE',  ( -69.03645266834649874, -271.6342739652374121, -202.5571738175895860 ) ) ;
#11342=CARTESIAN_POINT ( 'NONE',  ( -97.45849390208093155, -275.0761269559565676, -226.3745845701654389 ) ) ;
#11343=CARTESIAN_POINT ( 'NONE',  ( -111.7772303698380654, -288.6214340210744353, -271.1772261372534558 ) ) ;
#11344=CARTESIAN_POINT ( 'NONE',  ( -39.89717350363931558, -278.9443156487969873, -346.0956694798783246 ) ) ;
#11346=CARTESIAN_POINT ( 'NONE',  ( 18.83610338561120656, -280.8908376603206989, -223.7256858430666853 ) ) ;
#11347=CARTESIAN_POINT ( 'NONE',  ( 33.21414182896251788, -280.6478811249043019, -251.1882004953533283 ) ) ;
#11348=CARTESIAN_POINT ( 'NONE',  ( -6.685583423570927941, -277.7387027321283313, -340.6725089521601149 ) ) ;
#11349=CARTESIAN_POINT ( 'NONE',  ( -11.62811137551423535, -279.1745028002294475, -198.1471210626963568 ) ) ;
#11351=CARTESIAN_POINT ( 'NONE',  ( 166.0636734013047260, 231.1879126283853907, -190.4032150769705822 ) ) ;
#11352=CARTESIAN_POINT ( 'NONE',  ( -0.1699131758216758381, -275.4753885196952297, -203.1816090986692416 ) ) ;
#11354=CARTESIAN_POINT ( 'NONE',  ( -29.92569908550941093, -275.6645291668938853, -194.4156725579751992 ) ) ;
#11355=CARTESIAN_POINT ( 'NONE',  ( -95.99890600148557951, -299.6948066931273615, -223.6242672951989618 ) ) ;
#11358=CARTESIAN_POINT ( 'NONE',  ( 34.86946505646591987, -288.4620281699108659, -257.4349115767386138 ) ) ;
#11359=CARTESIAN_POINT ( 'NONE',  ( 4.601412699341469015, -288.3695778352252432, -206.9364085998001883 ) ) ;
#11360=CARTESIAN_POINT ( 'NONE',  ( -109.7250503732969804, -289.7648599649226071, -280.6756346987486381 ) ) ;
#11362=CARTESIAN_POINT ( 'NONE',  ( 26.30998212857352669, -286.4892510101543621, -227.1173277260599548 ) ) ;
#11364=CARTESIAN_POINT ( 'NONE',  ( 1.505277314044181525, -280.9238368440570639, -333.1691106938492908 ) ) ;
#11365=CARTESIAN_POINT ( 'NONE',  ( -0.3558064006185132078, -290.4156692189535534, -334.7857317213698138 ) ) ;
#11366=CARTESIAN_POINT ( 'NONE',  ( -85.32777244585830090, -282.2094553273086035, -326.2900426472295976 ) ) ;
#11368=CARTESIAN_POINT ( 'NONE',  ( -110.8853594847917776, -279.8634613372489639, -270.6566394101948845 ) ) ;
#11369=CARTESIAN_POINT ( 'NONE',  ( -18.99544303858672833, -277.3018856978719100, -341.0817181798996103 ) ) ;
#11370=CARTESIAN_POINT ( 'NONE',  ( -109.0964789659408751, -289.6897383788099773, -243.3910039210418006 ) ) ;
#11372=CARTESIAN_POINT ( 'NONE',  ( -109.8283219981287857, -285.6772374939705514, -244.8689923333030265 ) ) ;
#11373=CARTESIAN_POINT ( 'NONE',  ( -78.49484393398729765, -286.0062345702976927, -205.3538440969740861 ) ) ;
#11374=CARTESIAN_POINT ( 'NONE',  ( 21.01118224543156998, -282.3349793459746593, -314.2445284700164621 ) ) ;
#11377=CARTESIAN_POINT ( 'NONE',  ( -85.74245417775968292, -293.2512084317741596, -212.0034216803959737 ) ) ;
#11378=CARTESIAN_POINT ( 'NONE',  ( 31.77725959581172077, -292.6614447000270047, -303.2849806446945422 ) ) ;
#11379=CARTESIAN_POINT ( 'NONE',  ( -29.95425096144462529, -273.2066927464597939, -197.4993718956545194 ) ) ;
#11380=CARTESIAN_POINT ( 'NONE',  ( -113.5527564093087278, -295.7674166560302638, -281.0075193327135707 ) ) ;
#11381=CARTESIAN_POINT ( 'NONE',  ( -55.16144963479948871, -290.2986411969301344, -198.8547247155877074 ) ) ;
#11382=CARTESIAN_POINT ( 'NONE',  ( -35.64961170260739465, -293.2705259172656156, -344.3677798217680674 ) ) ;
#11383=CARTESIAN_POINT ( 'NONE',  ( -105.4759555427107358, -291.3922999811293266, -297.7894596594096583 ) ) ;
#11385=CARTESIAN_POINT ( 'NONE',  ( 36.55020258979707393, -291.7294831565670279, -284.2151388565059733 ) ) ;
#11386=CARTESIAN_POINT ( 'NONE',  ( -55.96901422286584449, -297.2920558577019960, -343.0641538239559054 ) ) ;
#11387=CARTESIAN_POINT ( 'NONE',  ( -87.86546529836977015, -286.2657948846150475, -217.3445394364528909 ) ) ;
#11388=CARTESIAN_POINT ( 'NONE',  ( 37.98597651331754577, -277.5060199872726798, -268.3244708241073226 ) ) ;
#11389=CARTESIAN_POINT ( 'NONE',  ( -107.2202210201238017, -276.9427204500062203, -301.8749748085886040 ) ) ;
#11390=CARTESIAN_POINT ( 'NONE',  ( -34.75589845781152576, -297.2809260219823386, -193.5229350376594084 ) ) ;
#11391=CARTESIAN_POINT ( 'NONE',  ( 23.28315414248127624, -274.3770698639895613, -312.9061203951491166 ) ) ;
#11392=CARTESIAN_POINT ( 'NONE',  ( -94.17406662523710281, -277.3022651727242192, -222.2645355134858960 ) ) ;
#11393=CARTESIAN_POINT ( 'NONE',  ( -56.98255259209989276, -274.9983418301884512, -199.5877651041261345 ) ) ;
#11394=CARTESIAN_POINT ( 'NONE',  ( -97.31204832372311841, -276.3170232525630468, -317.3717312079050430 ) ) ;
#11396=CARTESIAN_POINT ( 'NONE',  ( -81.13870037973701699, -274.0908838076598499, -211.7679830997394959 ) ) ;
#11397=DIRECTION ( 'NONE',  ( 0.000000000000000000, 1.000000000000000000, -1.224646799147353207E-16 ) ) ;
#11398=CARTESIAN_POINT ( 'NONE',  ( -64.87016117494248135, -287.4298902250495189, -340.5631881141715667 ) ) ;
#11399=CARTESIAN_POINT ( 'NONE',  ( -11.48823446740222032, -274.2317006526435534, -202.0384963232974940 ) ) ;
#11400=CARTESIAN_POINT ( 'NONE',  ( 36.78441279345251758, -287.8138627200721089, -291.2498027762903234 ) ) ;
#11401=CARTESIAN_POINT ( 'NONE',  ( -69.35238401008209053, -289.1286462285888206, -340.3831119873746047 ) ) ;
#11402=CARTESIAN_POINT ( 'NONE',  ( -40.39932015838823531, -299.9939157610626239, -195.0169606266555036 ) ) ;
#11403=CARTESIAN_POINT ( 'NONE',  ( 28.76599078492039396, -292.0193218058253137, -305.5403066563320635 ) ) ;
#11404=CARTESIAN_POINT ( 'NONE',  ( 37.52249607088534589, -280.5317742177047649, -252.9968900744329972 ) ) ;
#11405=CARTESIAN_POINT ( 'NONE',  ( 22.68542923180448057, -296.3033736090878278, -195.3865787154307441 ) ) ;
#11406=CARTESIAN_POINT ( 'NONE',  ( -93.73448883533198739, -277.2394758535182291, -220.8395359513654057 ) ) ;
#11408=CARTESIAN_POINT ( 'NONE',  ( 19.81307960487046316, -286.9946250090910667, -316.4095887485784147 ) ) ;
#11411=CARTESIAN_POINT ( 'NONE',  ( -58.18703868680834290, -289.7827586610171693, -198.2618640257711604 ) ) ;
#11412=CARTESIAN_POINT ( 'NONE',  ( 22.83592406990304013, -276.4838422028288960, -227.8026935853109762 ) ) ;
#11413=CARTESIAN_POINT ( 'NONE',  ( 38.94217531313751834, -283.0434760568230104, -275.6022591515587692 ) ) ;
#11414=CARTESIAN_POINT ( 'NONE',  ( -36.18977776368984678, -296.0866170971119686, -195.0062959027168006 ) ) ;
#11415=CARTESIAN_POINT ( 'NONE',  ( -110.3187896272780932, -284.5089228646999118, -273.6381354138727033 ) ) ;
#11416=CARTESIAN_POINT ( 'NONE',  ( 21.94520876119978681, -276.3714986951895867, -226.7671120568137439 ) ) ;
#11417=CARTESIAN_POINT ( 'NONE',  ( 34.27732038458702135, -276.1574838319912146, -255.3561829670659620 ) ) ;
#11418=CARTESIAN_POINT ( 'NONE',  ( -57.91307169582564285, -285.3178921301194464, -342.5388085858872387 ) ) ;
#11419=CARTESIAN_POINT ( 'NONE',  ( -74.41789684930030546, -272.4672874572282240, -207.0600733800549165 ) ) ;
#11421=CARTESIAN_POINT ( 'NONE',  ( 202.9738562182569694, 291.9636489450776367, -53.99999999998589573 ) ) ;
#11422=CARTESIAN_POINT ( 'NONE',  ( -24.90990485622979023, -294.7312330327834502, -346.4049884760342479 ) ) ;
#11423=CARTESIAN_POINT ( 'NONE',  ( -110.3230030974495719, -286.3290913668477629, -286.0926037668029380 ) ) ;
#11425=CARTESIAN_POINT ( 'NONE',  ( 99.50465036329318025, -297.2649936051624309, -195.4191791630918829 ) ) ;
#11426=CARTESIAN_POINT ( 'NONE',  ( -80.14473762126785061, -276.8124489957585865, -334.2378595661368195 ) ) ;
#11427=CARTESIAN_POINT ( 'NONE',  ( -113.3165986411326571, -288.8698335051075219, -276.8648168246490968 ) ) ;
#11428=CARTESIAN_POINT ( 'NONE',  ( -8.202442798970212223, -284.1835824435787572, -338.0487197718591688 ) ) ;
#11430=CARTESIAN_POINT ( 'NONE',  ( -69.67412546411621577, -279.2438419996188941, -336.9528315824991864 ) ) ;
#11431=CARTESIAN_POINT ( 'NONE',  ( -107.3932622177593004, -286.3709757065608414, -239.7101484561688949 ) ) ;
#11432=CARTESIAN_POINT ( 'NONE',  ( 19.46310423882188445, -282.8732092315353839, -221.3698402362720117 ) ) ;
#11433=CARTESIAN_POINT ( 'NONE',  ( 29.94649989121425193, -275.2323519110170764, -232.8175652762110985 ) ) ;
#11434=CARTESIAN_POINT ( 'NONE',  ( -96.15056425276520713, -277.7156232632123647, -320.0857701678258991 ) ) ;
#11436=CARTESIAN_POINT ( 'NONE',  ( -108.2332687382704819, -298.1750230079541666, -293.2368349063028177 ) ) ;
#11439=CARTESIAN_POINT ( 'NONE',  ( 51.79982928851320878, -297.2963346967968619, -194.6241899864013192 ) ) ;
#11440=CARTESIAN_POINT ( 'NONE',  ( 29.20774096101851924, -275.4658549147889062, -300.5134036702175990 ) ) ;
#11441=CARTESIAN_POINT ( 'NONE',  ( -34.07718661552963368, -299.1717895042510236, -193.6696448167754454 ) ) ;
#11442=CARTESIAN_POINT ( 'NONE',  ( -4.160082858052456700, -288.2559950131039841, -204.2025638000948504 ) ) ;
#11443=CARTESIAN_POINT ( 'NONE',  ( -36.26464106556716160, -296.5590312381929721, -346.6731709522434812 ) ) ;
#11444=CARTESIAN_POINT ( 'NONE',  ( -111.5800121149757160, -297.5190723850998324, -289.3000501851827835 ) ) ;
#11445=CARTESIAN_POINT ( 'NONE',  ( -109.4866115917095897, -292.2938767789697749, -290.4299665183043544 ) ) ;
#11446=CARTESIAN_POINT ( 'NONE',  ( -62.91204080322021497, -277.7184462700200243, -199.9773019534132743 ) ) ;
#11447=CARTESIAN_POINT ( 'NONE',  ( -110.3034457167512414, -280.6640958970323254, -255.5356416199172145 ) ) ;
#11448=CARTESIAN_POINT ( 'NONE',  ( -47.44444569349431617, -296.0027431062397341, -196.5576365706783406 ) ) ;
#11449=CARTESIAN_POINT ( 'NONE',  ( -30.30563378287073562, -284.8244523437048201, -345.7985042736161745 ) ) ;
#11450=CARTESIAN_POINT ( 'NONE',  ( 34.30100721949369813, -286.2683203468890838, -254.8192854472428053 ) ) ;
#11451=CARTESIAN_POINT ( 'NONE',  ( -29.52244597877754373, -125.2720606855327645, -363.9572059679637164 ) ) ;
#11453=CARTESIAN_POINT ( 'NONE',  ( -39.97043042295008064, -285.6849327779158898, -197.3873058039590092 ) ) ;
#11455=CARTESIAN_POINT ( 'NONE',  ( -58.38866193284027872, -284.3975512039889963, -344.1626984338965372 ) ) ;
#11456=CARTESIAN_POINT ( 'NONE',  ( -74.28774443070166456, -273.8800120937729616, -207.3178043428175386 ) ) ;
#11457=CARTESIAN_POINT ( 'NONE',  ( 37.63803112149120267, -286.1490916994732743, -254.6116087331639619 ) ) ;
#11458=CARTESIAN_POINT ( 'NONE',  ( -19.82160859362019067, -281.2131800830991324, -195.5678616846588227 ) ) ;
#11461=CARTESIAN_POINT ( 'NONE',  ( -95.39107686109805684, -280.7465174123743736, -220.8134983719806144 ) ) ;
#11462=CARTESIAN_POINT ( 'NONE',  ( 12.97514498431736030, -281.0660220433105110, -212.1034198699930755 ) ) ;
#11463=CARTESIAN_POINT ( 'NONE',  ( -6.941161984400256557, -283.9809262143061233, -207.3071070584150277 ) ) ;
#11464=CARTESIAN_POINT ( 'NONE',  ( 85.12579728816612601, 83.07458439776537773, -302.4277712846086388 ) ) ;
#11466=CARTESIAN_POINT ( 'NONE',  ( -27.06294769334709471, -276.1831539464841399, -196.1848865931888497 ) ) ;
#11467=CARTESIAN_POINT ( 'NONE',  ( -84.62815394613997455, -219.0928880101756704, -352.2053832115043974 ) ) ;
#11468=CARTESIAN_POINT ( 'NONE',  ( 20.97651499013447207, -278.9285694221537142, -223.7689234350514766 ) ) ;
#11469=CARTESIAN_POINT ( 'NONE',  ( 35.72353641092399101, -295.0466737807587947, -249.4464324571203235 ) ) ;
#11470=CARTESIAN_POINT ( 'NONE',  ( -107.7031715467910260, -295.6389931028600131, -290.1892799794342750 ) ) ;
#11471=CARTESIAN_POINT ( 'NONE',  ( -4.624614936613887117, -291.9793798705346717, -200.7255003711733821 ) ) ;
#11472=CARTESIAN_POINT ( 'NONE',  ( -104.9195836729377191, -260.6502345264863720, -315.6181490027343557 ) ) ;
#11473=CARTESIAN_POINT ( 'NONE',  ( -111.0488184132014311, -295.3833861899994417, -250.0196381538110018 ) ) ;
#11474=CARTESIAN_POINT ( 'NONE',  ( 36.07227124826489018, -285.8536498959455798, -262.8226021462563722 ) ) ;
#11475=CARTESIAN_POINT ( 'NONE',  ( 18.01723649435033181, -296.1084460155602187, -319.8399065829707979 ) ) ;
#11476=CARTESIAN_POINT ( 'NONE',  ( 32.74892890134105272, -285.9454472552562265, -248.2158515072573266 ) ) ;
#11477=CARTESIAN_POINT ( 'NONE',  ( -90.02799977710412804, -286.6039323911152792, -219.0494396915206039 ) ) ;
#11479=CARTESIAN_POINT ( 'NONE',  ( 38.58559150408168392, -294.6352542864493671, -281.6689293700790699 ) ) ;
#11480=CARTESIAN_POINT ( 'NONE',  ( -1.216129416510071115, -283.0512547400093695, -333.8664845470268006 ) ) ;
#11481=CARTESIAN_POINT ( 'NONE',  ( -92.42221285259176966, -294.6140288385988697, -323.5978143141338137 ) ) ;
#11482=CARTESIAN_POINT ( 'NONE',  ( -106.3639559085468704, -290.9191095673795076, -304.2472036212384410 ) ) ;
#11483=CARTESIAN_POINT ( 'NONE',  ( -4.636001466699962492, -292.9639148862775073, -200.7201517441747001 ) ) ;
#11484=CARTESIAN_POINT ( 'NONE',  ( -39.95589968992072016, -289.2524614877446538, -343.3638723023991588 ) ) ;
#11487=CARTESIAN_POINT ( 'NONE',  ( -103.5123887959996409, -297.9251030542459375, -307.3701453069767808 ) ) ;
#11488=CARTESIAN_POINT ( 'NONE',  ( 98.11687111328420485, -298.3994096029719003, -193.8837290502138160 ) ) ;
#11490=CARTESIAN_POINT ( 'NONE',  ( -5.445217454625628228, -279.5411907961400289, -204.4367458427530266 ) ) ;
#11491=CARTESIAN_POINT ( 'NONE',  ( -5.134309819086812610, -273.9724995160595427, -200.4882984245600994 ) ) ;
#11492=CARTESIAN_POINT ( 'NONE',  ( -69.54318831975241721, -296.1002413525507677, -204.0755847722494423 ) ) ;
#11493=CARTESIAN_POINT ( 'NONE',  ( -81.53605894583266434, -279.5212305605182337, -330.0077786293063582 ) ) ;
#11494=CARTESIAN_POINT ( 'NONE',  ( 36.83490362576873167, -273.7441626959432597, -274.4031117153029413 ) ) ;
#11495=CARTESIAN_POINT ( 'NONE',  ( -6.584612420995379800, -295.8440838470920653, -337.0029371490374501 ) ) ;
#11496=CARTESIAN_POINT ( 'NONE',  ( -105.0529562735668208, -298.0070062402089093, -242.2646437551103702 ) ) ;
#11498=CARTESIAN_POINT ( 'NONE',  ( -113.3248288483426762, -298.2331975103411992, -263.9581772851617529 ) ) ;
#11499=CARTESIAN_POINT ( 'NONE',  ( -36.53874163567517996, -296.0620253656962291, -195.1947156145810425 ) ) ;
#11500=CARTESIAN_POINT ( 'NONE',  ( 14.39427520030632657, -294.9526403546959159, -322.0780313726114628 ) ) ;
#11501=CARTESIAN_POINT ( 'NONE',  ( -104.0831550980230418, -289.5419824366031207, -239.3618743800400637 ) ) ;
#11503=CARTESIAN_POINT ( 'NONE',  ( -3.858559478608783788, -274.9743928494764873, -201.0760927360696257 ) ) ;
#11504=CARTESIAN_POINT ( 'NONE',  ( -35.15122092426700817, -298.4135995138944395, -197.3398456385576765 ) ) ;
#11505=CARTESIAN_POINT ( 'NONE',  ( -6.113629538847954237, -284.6237049131701156, -338.9411035002154335 ) ) ;
#11507=CARTESIAN_POINT ( 'NONE',  ( -35.92522793467507114, -281.7196016093114395, -346.8678886647937816 ) ) ;
#11509=CARTESIAN_POINT ( 'NONE',  ( -41.38738884441230681, -276.4503954261335821, -347.1658790889136412 ) ) ;
#11510=CARTESIAN_POINT ( 'NONE',  ( -67.86102795488912420, -282.6604924618716268, -336.8530149059919268 ) ) ;
#11511=CARTESIAN_POINT ( 'NONE',  ( -14.01563164195555977, -280.7500629060195934, -341.8168592057301112 ) ) ;
#11512=CARTESIAN_POINT ( 'NONE',  ( 33.43168896984582972, -273.8602827569240503, -250.0169715893742364 ) ) ;
#11513=CARTESIAN_POINT ( 'NONE',  ( -59.57981250831698361, -279.3401748849400406, -342.0421395490499776 ) ) ;
#11516=CARTESIAN_POINT ( 'NONE',  ( -36.88163231859655156, -296.2977026140270596, -194.3745803279026916 ) ) ;
#11517=CARTESIAN_POINT ( 'NONE',  ( -106.8278119566251831, -280.9255136185743709, -241.6956564145168329 ) ) ;
#11519=CARTESIAN_POINT ( 'NONE',  ( -112.9138559037067182, -286.4408799082561359, -272.8270985848679402 ) ) ;
#11522=CARTESIAN_POINT ( 'NONE',  ( 12.56710903178727534, -286.3568403398864461, -326.4130420163684221 ) ) ;
#11524=CARTESIAN_POINT ( 'NONE',  ( -95.59490051737277838, -295.9720864045256121, -225.6898309268584626 ) ) ;
#11525=CARTESIAN_POINT ( 'NONE',  ( -53.70344102723436208, -287.4039243361898457, -342.7707783337318119 ) ) ;
#11526=CARTESIAN_POINT ( 'NONE',  ( -53.17117378510891967, -153.5335516589311737, -364.2630158522994179 ) ) ;
#11527=CARTESIAN_POINT ( 'NONE',  ( -110.5494919696190408, -294.3427326947924030, -286.6589665262314952 ) ) ;
#11528=CARTESIAN_POINT ( 'NONE',  ( -98.77442992329163474, -283.6398623706434137, -225.0113347756494022 ) ) ;
#11529=CARTESIAN_POINT ( 'NONE',  ( 15.82168780366188088, -282.4204734350224157, -219.1012770998071346 ) ) ;
#11530=CARTESIAN_POINT ( 'NONE',  ( -33.13751901158030222, -281.2397787458382936, -346.2443568781510521 ) ) ;
#11531=CARTESIAN_POINT ( 'NONE',  ( -72.35886167263529956, -289.5293361712776914, -334.4142084416675402 ) ) ;
#11532=CARTESIAN_POINT ( 'NONE',  ( -94.40887490260023185, -280.6297944397164770, -223.8991713785771651 ) ) ;
#11533=CARTESIAN_POINT ( 'NONE',  ( -66.14266353455525405, -280.4681358479791129, -203.0934053111797937 ) ) ;
#11534=CARTESIAN_POINT ( 'NONE',  ( 36.40842415022844847, -289.3335443232876401, -254.8285740615326915 ) ) ;
#11536=CARTESIAN_POINT ( 'NONE',  ( -110.1018633137572920, -272.8698358982286436, -245.1627320581836500 ) ) ;
#11537=CARTESIAN_POINT ( 'NONE',  ( -110.5469674573932366, -292.3429909457438498, -285.0152747344441764 ) ) ;
#11539=CARTESIAN_POINT ( 'NONE',  ( 25.22466315766300227, -290.6948066931273047, -320.2154176792147382 ) ) ;
#11541=CARTESIAN_POINT ( 'NONE',  ( 0.1109106937538962556, -274.5550432051274470, -335.5916923982401840 ) ) ;
#11543=CARTESIAN_POINT ( 'NONE',  ( -14.04619081289553506, -293.1547460610950111, -342.9128902544452444 ) ) ;
#11544=CARTESIAN_POINT ( 'NONE',  ( -44.56893824619808697, -297.4660286304355736, -197.6074923732301443 ) ) ;
#11545=CARTESIAN_POINT ( 'NONE',  ( -50.85983175033088344, -290.7479861537665329, -342.8561444416225186 ) ) ;
#11546=CARTESIAN_POINT ( 'NONE',  ( -36.15511286537676483, -284.7972155504232887, -344.3649423895672612 ) ) ;
#11547=CARTESIAN_POINT ( 'NONE',  ( -101.2015815193663144, -292.5343043824975666, -228.3075643155002581 ) ) ;
#11548=CARTESIAN_POINT ( 'NONE',  ( -40.62810733174035249, -293.3268314184469432, -193.9117867469470582 ) ) ;
#11549=CARTESIAN_POINT ( 'NONE',  ( -10.04516407786696952, -288.4086670894283770, -200.4909443072115494 ) ) ;
#11550=CARTESIAN_POINT ( 'NONE',  ( 1.372136844239459919, -280.7207461174638183, -203.7403742711566395 ) ) ;
#11551=CARTESIAN_POINT ( 'NONE',  ( -98.85080414034196394, -294.0386249543082613, -314.3348645217753869 ) ) ;
#11552=CARTESIAN_POINT ( 'NONE',  ( 17.82479500166395781, -282.1226721011521477, -324.1556216165811861 ) ) ;
#11553=CARTESIAN_POINT ( 'NONE',  ( 5.876947330639362477, -276.5050727388298810, -209.9402126790755290 ) ) ;
#11554=CARTESIAN_POINT ( 'NONE',  ( -21.33282851196159058, -279.3376638359844719, -340.3538533559490702 ) ) ;
#11555=CARTESIAN_POINT ( 'NONE',  ( -45.53989364634736603, -275.2944363086901376, -345.7332774168204423 ) ) ;
#11557=CARTESIAN_POINT ( 'NONE',  ( 9.943755245608874915, -281.8879246674198384, -326.1239116657922636 ) ) ;
#11558=CARTESIAN_POINT ( 'NONE',  ( -31.46533377740031412, -278.1847185798686155, -346.7906720702263215 ) ) ;
#11559=CARTESIAN_POINT ( 'NONE',  ( -2.319525372208536496, -285.5628516571409818, -202.0363260972031867 ) ) ;
#11560=CARTESIAN_POINT ( 'NONE',  ( 23.40701951457631935, -294.7307829323729038, -228.0591670476086108 ) ) ;
#11561=CARTESIAN_POINT ( 'NONE',  ( 28.41597052308757299, -277.6586671755612770, -308.8626655423060470 ) ) ;
#11562=CARTESIAN_POINT ( 'NONE',  ( 4.578856692953886309, -275.9199632546058183, -206.2985416266020025 ) ) ;
#11563=CARTESIAN_POINT ( 'NONE',  ( 0.8696174200904051022, -276.3605945279220464, -332.6209571198442063 ) ) ;
#11564=CARTESIAN_POINT ( 'NONE',  ( -74.18334530882417255, -297.5432225595473028, -335.4972953945558629 ) ) ;
#11565=CARTESIAN_POINT ( 'NONE',  ( -24.81035568559763504, -284.2120783810746047, -196.5318811778817576 ) ) ;
#11566=CARTESIAN_POINT ( 'NONE',  ( 32.16869925652592599, -292.7933900766773831, -237.1608193483886851 ) ) ;
#11567=CARTESIAN_POINT ( 'NONE',  ( -8.516674468338223392, -290.2812446754635403, -340.9128753623573402 ) ) ;
#11568=CARTESIAN_POINT ( 'NONE',  ( 26.51052486730400659, -291.9803529021078816, -234.2418894663271089 ) ) ;
#11570=CARTESIAN_POINT ( 'NONE',  ( -90.36389935942597162, -289.8944950071613675, -215.2672263030509328 ) ) ;
#11571=CARTESIAN_POINT ( 'NONE',  ( -1.242531588920580132, -292.2119008737589638, -206.8727260103918013 ) ) ;
#11573=CARTESIAN_POINT ( 'NONE',  ( -98.77324533424825859, -291.0183084803539373, -316.2920635262997280 ) ) ;
#11574=CARTESIAN_POINT ( 'NONE',  ( -109.0632492248754914, -278.7036895740114346, -284.1423713981456558 ) ) ;
#11575=CARTESIAN_POINT ( 'NONE',  ( -112.2954467929809255, -295.6770092014780289, -254.0693990215986844 ) ) ;
#11576=CARTESIAN_POINT ( 'NONE',  ( -49.33702200896129852, -286.5546397482127077, -194.3507213057398815 ) ) ;
#11578=CARTESIAN_POINT ( 'NONE',  ( 38.26861755794667630, -287.7046555250698248, -255.9103688320375909 ) ) ;
#11579=CARTESIAN_POINT ( 'NONE',  ( -101.0118354170628834, -285.3757170552138973, -234.5055412121603240 ) ) ;
#11580=CARTESIAN_POINT ( 'NONE',  ( -64.04501568489942542, -182.5871740903956209, -362.3045948285029567 ) ) ;
#11581=CARTESIAN_POINT ( 'NONE',  ( -113.0704522964411183, -269.5540774813418921, -295.9878753163457077 ) ) ;
#11582=CARTESIAN_POINT ( 'NONE',  ( 195.7885930606527438, 282.2018346885278106, -110.2488485752002418 ) ) ;
#11584=CARTESIAN_POINT ( 'NONE',  ( 32.24862845876810979, -275.0482150385315663, -292.9396009730232890 ) ) ;
#11585=CARTESIAN_POINT ( 'NONE',  ( 7.759790988737595541, -275.3402858988699791, -328.2192316810764510 ) ) ;
#11586=CARTESIAN_POINT ( 'NONE',  ( -75.74374658687683848, -297.0619129554684150, -203.6305705875854528 ) ) ;
#11587=CARTESIAN_POINT ( 'NONE',  ( 203.7386562182570060, 292.1033822784109475, -53.99999999998943423 ) ) ;
#11588=CARTESIAN_POINT ( 'NONE',  ( 37.46674707484939404, -274.0344211875304268, -254.2680747095361653 ) ) ;
#11589=CARTESIAN_POINT ( 'NONE',  ( 97.19193867083082239, -301.6141606055674060, -196.0827732276452480 ) ) ;
#11590=CARTESIAN_POINT ( 'NONE',  ( -33.36172283956069862, -299.0420852247531798, -193.5957918784854712 ) ) ;
#11591=CARTESIAN_POINT ( 'NONE',  ( -13.26168312770531088, -289.2230987187677442, -339.3403990955671361 ) ) ;
#11592=CARTESIAN_POINT ( 'NONE',  ( -64.20014745993481142, -296.1966677711534999, -342.3526635091344019 ) ) ;
#11593=CARTESIAN_POINT ( 'NONE',  ( -46.12907256121117427, -298.4358671745771971, -193.9261195272139844 ) ) ;
#11594=CARTESIAN_POINT ( 'NONE',  ( -5.539589312092116025, -294.7884655921533863, -336.0835717210860025 ) ) ;
#11596=CARTESIAN_POINT ( 'NONE',  ( 34.35566330565874438, -277.1644542615528053, -246.3467742006522769 ) ) ;
#11600=CARTESIAN_POINT ( 'NONE',  ( -59.27859297360825508, -279.2832248190913447, -196.6162901275342278 ) ) ;
#11602=CARTESIAN_POINT ( 'NONE',  ( -51.31407577090775618, -278.1764662041657630, -342.2511810393753535 ) ) ;
#11603=CARTESIAN_POINT ( 'NONE',  ( -3.160588105494891664, -278.3671081626870887, -338.2403641731778521 ) ) ;
#11604=CARTESIAN_POINT ( 'NONE',  ( -102.2031762563668309, -276.0604935216273361, -308.8222777740136280 ) ) ;
#11605=CARTESIAN_POINT ( 'NONE',  ( -96.33476895739782719, -273.6485508082550382, -227.1747776428907173 ) ) ;
#11606=CARTESIAN_POINT ( 'NONE',  ( -44.60935979190379896, -296.5332539400791347, -197.0808543419433647 ) ) ;
#11608=CARTESIAN_POINT ( 'NONE',  ( -106.2635040667686610, -278.3969885493340826, -294.5723588836564772 ) ) ;
#11609=CARTESIAN_POINT ( 'NONE',  ( -12.40042463954857332, -287.4193648854037519, -342.7438763495526928 ) ) ;
#11610=CARTESIAN_POINT ( 'NONE',  ( -36.97575334906754563, -276.0569231635925576, -195.3492938116267226 ) ) ;
#11612=CARTESIAN_POINT ( 'NONE',  ( -75.96263931986773343, -288.7796748299530236, -332.4982629346425824 ) ) ;
#11613=CARTESIAN_POINT ( 'NONE',  ( -94.32919781409560755, -283.1982718715816532, -322.0114345590041580 ) ) ;
#11614=CARTESIAN_POINT ( 'NONE',  ( 6.169978848331856724, -280.6922266477875496, -330.2335473955945417 ) ) ;
#11615=CARTESIAN_POINT ( 'NONE',  ( 35.15064247038245071, -279.9612275208723418, -257.7027143469986754 ) ) ;
#11616=CARTESIAN_POINT ( 'NONE',  ( -109.4169125134991134, -282.8729681504414657, -251.7471995278742156 ) ) ;
#11617=CARTESIAN_POINT ( 'NONE',  ( -25.03178290578624399, -288.2091696749959624, -196.3264024738879243 ) ) ;
#11618=CARTESIAN_POINT ( 'NONE',  ( -102.2006786956894757, -279.2917446365155456, -304.7186994294927445 ) ) ;
#11620=CARTESIAN_POINT ( 'NONE',  ( -80.79295932109633327, -293.4626542217836800, -209.2302033757691788 ) ) ;
#11621=CARTESIAN_POINT ( 'NONE',  ( -96.28278228896346036, -276.1397277320244825, -318.3390113488942461 ) ) ;
#11622=CARTESIAN_POINT ( 'NONE',  ( 25.46738383376368020, -276.7170583646852151, -307.7631451985898821 ) ) ;
#11623=CARTESIAN_POINT ( 'NONE',  ( -108.9314939596393543, -286.2567375103013774, -293.3148658332976311 ) ) ;
#11625=CARTESIAN_POINT ( 'NONE',  ( -106.4050623250753915, -292.0721932180657632, -301.1420541801509216 ) ) ;
#11626=CARTESIAN_POINT ( 'NONE',  ( -111.4131706052021826, -294.3998911031088710, -282.2070421955319830 ) ) ;
#11627=CARTESIAN_POINT ( 'NONE',  ( -12.74570201443743223, -285.5611213048340460, -197.5655432750447744 ) ) ;
#11628=CARTESIAN_POINT ( 'NONE',  ( -110.0615381874820429, -289.1199781494431704, -257.4894350983458366 ) ) ;
#11629=CARTESIAN_POINT ( 'NONE',  ( 82.64890176555634582, -299.5541904835127980, -202.0153591320744226 ) ) ;
#11630=CARTESIAN_POINT ( 'NONE',  ( 29.59658498552832029, -274.6431605175964705, -300.7010168396257086 ) ) ;
#11631=CARTESIAN_POINT ( 'NONE',  ( 17.04827757031210211, -292.4058820509746397, -320.8843384530421758 ) ) ;
#11633=CARTESIAN_POINT ( 'NONE',  ( 144.2857639756989272, -299.5541904835127980, -195.3611179825600175 ) ) ;
#11634=CARTESIAN_POINT ( 'NONE',  ( -64.12712969097799487, -290.1889964378135573, -198.8544353375396838 ) ) ;
#11635=CARTESIAN_POINT ( 'NONE',  ( -98.78428046866444845, -286.7136077545509352, -229.4801965607597367 ) ) ;
#11636=CARTESIAN_POINT ( 'NONE',  ( 29.46100516558870908, -286.2679947538612737, -306.6839816260460339 ) ) ;
#11637=CARTESIAN_POINT ( 'NONE',  ( -105.1474911294664878, -286.3597133522752074, -241.6337416539681726 ) ) ;
#11639=CARTESIAN_POINT ( 'NONE',  ( -60.03840806735935587, -286.5531606275172862, -200.8092583711334100 ) ) ;
#11640=CARTESIAN_POINT ( 'NONE',  ( 32.91987177790567642, -295.1778266320673083, -242.9825372491910969 ) ) ;
#11641=CARTESIAN_POINT ( 'NONE',  ( -88.26010818284377990, -275.8386055020574759, -326.1879029240238310 ) ) ;
#11642=CARTESIAN_POINT ( 'NONE',  ( -5.289708302656784156, -276.9750615321442524, -340.3497892919464221 ) ) ;
#11643=CARTESIAN_POINT ( 'NONE',  ( 16.48136691980723256, -290.8891718643524200, -217.2554290598356488 ) ) ;
#11644=CARTESIAN_POINT ( 'NONE',  ( -111.3372469311076856, -278.8191976690511638, -249.0618444428088765 ) ) ;
#11645=CARTESIAN_POINT ( 'NONE',  ( -74.09069615543015175, -297.5229575377426841, -335.3330972860230759 ) ) ;
#11648=CARTESIAN_POINT ( 'NONE',  ( 32.31329700962663054, -285.9276872772892375, -246.9213045967846654 ) ) ;
#11649=CARTESIAN_POINT ( 'NONE',  ( -108.3042741779299689, -276.4057819892398129, -292.3320249914052056 ) ) ;
#11650=CARTESIAN_POINT ( 'NONE',  ( 25.04376588432860018, -280.1146008827191167, -311.9910865051884912 ) ) ;
#11651=DIRECTION ( 'NONE',  ( 0.000000000000000000, 0.000000000000000000, 1.000000000000000000 ) ) ;
#11652=CARTESIAN_POINT ( 'NONE',  ( -29.88718316410720632, -272.6247755084341406, -194.4194434616762237 ) ) ;
#11653=CARTESIAN_POINT ( 'NONE',  ( 36.33594807749791755, -295.1132910682781585, -273.4993714367753910 ) ) ;
#11654=CARTESIAN_POINT ( 'NONE',  ( 23.51046387246500302, -279.8471644805388223, -223.6651848667837044 ) ) ;
#11655=CARTESIAN_POINT ( 'NONE',  ( -3.022918825840486434, -295.5281451286790002, -335.0575606866904650 ) ) ;
#11656=CARTESIAN_POINT ( 'NONE',  ( -111.4865478233219278, -297.6291528604314749, -289.2776772275749977 ) ) ;
#11657=CARTESIAN_POINT ( 'NONE',  ( -41.86622181449494207, -297.8268698960334859, -197.5014672283679715 ) ) ;
#11658=CARTESIAN_POINT ( 'NONE',  ( -94.99312199470141138, -293.2149144762724973, -222.3690452327836056 ) ) ;
#11659=CARTESIAN_POINT ( 'NONE',  ( -73.61489112234414733, -285.7513802489950763, -202.3811118123230699 ) ) ;
#11660=CARTESIAN_POINT ( 'NONE',  ( 36.03645121284596087, -273.9317012814196346, -289.2278185178793706 ) ) ;
#11661=CARTESIAN_POINT ( 'NONE',  ( 18.64335908102332695, -288.1074178690261078, -323.2257862389564025 ) ) ;
#11663=CARTESIAN_POINT ( 'NONE',  ( 34.22849508360164350, -286.4067173510317730, -254.8332203058909045 ) ) ;
#11664=CARTESIAN_POINT ( 'NONE',  ( -66.22116472758847294, -289.6739569152180707, -201.1442329411145238 ) ) ;
#11666=CARTESIAN_POINT ( 'NONE',  ( -75.10193482699480683, -210.9688814900462432, -359.8487438039043127 ) ) ;
#11667=CARTESIAN_POINT ( 'NONE',  ( -70.00559712005777158, -289.0021050615021068, -335.7283235549663232 ) ) ;
#11669=CARTESIAN_POINT ( 'NONE',  ( -102.7114169038248264, -284.9657750020126059, -310.6056249522939083 ) ) ;
#11670=CARTESIAN_POINT ( 'NONE',  ( 37.55171220868359683, -292.8229808298123658, -287.2666842175201509 ) ) ;
#11671=CARTESIAN_POINT ( 'NONE',  ( 37.88141747907987167, -283.3070123656646047, -282.6051177324919195 ) ) ;
#11672=CARTESIAN_POINT ( 'NONE',  ( 24.18511593081843358, -282.2590850588985631, -224.8886078306695708 ) ) ;
#11673=CARTESIAN_POINT ( 'NONE',  ( -10.97775055176488834, -282.5321013339286651, -338.4877626633717682 ) ) ;
#11674=CARTESIAN_POINT ( 'NONE',  ( -24.27228820052091507, -276.2190463883545704, -196.4556234875636278 ) ) ;
#11675=CARTESIAN_POINT ( 'NONE',  ( -100.0085033970901378, -295.9584688961542156, -315.1932064507313953 ) ) ;
#11676=CARTESIAN_POINT ( 'NONE',  ( -111.9515173681788838, -288.5257767519766503, -273.9637530710510873 ) ) ;
#11677=CARTESIAN_POINT ( 'NONE',  ( -72.98519972288366375, -296.4882235488046263, -206.3004669503997945 ) ) ;
#11678=ORIENTED_EDGE ( 'NONE', *, *, #14901, .F. ) ;
#11681=CARTESIAN_POINT ( 'NONE',  ( -107.5233276065386150, -286.1466326648921950, -295.3308615078214530 ) ) ;
#11682=CARTESIAN_POINT ( 'NONE',  ( -33.43677011586752457, -296.0837740014431461, -346.9655942397035915 ) ) ;
#11683=CARTESIAN_POINT ( 'NONE',  ( -42.93244548060171439, -283.7758508834265285, -343.2991078337446424 ) ) ;
#11684=CARTESIAN_POINT ( 'NONE',  ( -34.31241549124833767, -276.0736885875668349, -347.0660307852529058 ) ) ;
#11685=CARTESIAN_POINT ( 'NONE',  ( -69.58799349518503163, -292.2901725061936418, -200.5364135441451481 ) ) ;
#11686=CARTESIAN_POINT ( 'NONE',  ( -57.40565113898599492, -283.9356145187182392, -197.2467975960159094 ) ) ;
#11687=CARTESIAN_POINT ( 'NONE',  ( -86.50279144521452679, -291.7243194107862791, -211.0556685650587383 ) ) ;
#11688=CARTESIAN_POINT ( 'NONE',  ( -109.7216608513759581, -291.0177183754245220, -260.3304151526854753 ) ) ;
#11691=CARTESIAN_POINT ( 'NONE',  ( 26.11126514475094140, -24.39807644324349667, -341.5406973817991343 ) ) ;
#11692=CARTESIAN_POINT ( 'NONE',  ( -34.48536626912725467, -284.5369755402188048, -346.6143088077583343 ) ) ;
#11693=CARTESIAN_POINT ( 'NONE',  ( -95.99890600148557951, -287.4094976428776249, -317.0979686699210447 ) ) ;
#11695=CARTESIAN_POINT ( 'NONE',  ( -1.111146971636954639, -281.4794899202430543, -334.0915902221684632 ) ) ;
#11696=CARTESIAN_POINT ( 'NONE',  ( 37.57030876805323771, -275.4411775086145440, -288.1360987535976506 ) ) ;
#11697=CARTESIAN_POINT ( 'NONE',  ( -90.80066947534646715, -281.2923472873845867, -217.9219484851064976 ) ) ;
#11698=CARTESIAN_POINT ( 'NONE',  ( -68.68430080596803577, -197.1092947213748801, -358.3343516210577491 ) ) ;
#11699=CARTESIAN_POINT ( 'NONE',  ( 31.85105581707266253, -280.5466157161601473, -302.9043616880563263 ) ) ;
#11700=CARTESIAN_POINT ( 'NONE',  ( -77.92258379212319142, -283.5245112615154994, -207.6496734141182117 ) ) ;
#11701=CARTESIAN_POINT ( 'NONE',  ( -34.12330758321979118, -299.8520531893593102, -194.3734957074033787 ) ) ;
#11702=CARTESIAN_POINT ( 'NONE',  ( -10.46153253366171754, -295.1840593404305082, -338.2981846826284027 ) ) ;
#11704=CARTESIAN_POINT ( 'NONE',  ( -109.9086964929104084, -289.0835355329542153, -282.0711414671125112 ) ) ;
#11705=CARTESIAN_POINT ( 'NONE',  ( 8.187397591614196557, -277.0993197920200259, -332.3981239670805508 ) ) ;
#11706=CARTESIAN_POINT ( 'NONE',  ( -19.27162332516118681, -274.2910648713669275, -199.5805329121355953 ) ) ;
#11707=CARTESIAN_POINT ( 'NONE',  ( 36.19314342898342574, -274.7472866812546499, -292.1817026711595418 ) ) ;
#11708=CARTESIAN_POINT ( 'NONE',  ( 133.0380396672494783, -299.5541904835127980, -195.3611179825600175 ) ) ;
#11709=CARTESIAN_POINT ( 'NONE',  ( -106.3021228730598295, -270.9389989292703831, -240.7440863109640077 ) ) ;
#11712=CARTESIAN_POINT ( 'NONE',  ( -16.02956128768343547, -283.8496364557395282, -340.5039637401467871 ) ) ;
#11713=CARTESIAN_POINT ( 'NONE',  ( -0.8422296462996153865, -284.3345153356459605, -337.0224127571835311 ) ) ;
#11714=CARTESIAN_POINT ( 'NONE',  ( -99.12161761480486177, -283.3603405406467459, -309.5344671044090887 ) ) ;
#11715=CARTESIAN_POINT ( 'NONE',  ( -56.83084584935117789, -275.7074002510711921, -341.5943448547106982 ) ) ;
#11716=CARTESIAN_POINT ( 'NONE',  ( -7.984325615633683704, -284.5238214239820991, -338.5447673707404874 ) ) ;
#11717=CARTESIAN_POINT ( 'NONE',  ( -37.83363503378704706, -275.5382638401135296, -344.0653827548361505 ) ) ;
#11720=CARTESIAN_POINT ( 'NONE',  ( -69.90327055032263104, -280.4370216824067370, -200.7486047600565087 ) ) ;
#11723=EDGE_LOOP ( 'NONE', ( #3891, #57612, #83619, #43939 ) ) ;
#11725=CARTESIAN_POINT ( 'NONE',  ( -91.04444654790594882, -287.1595835766373170, -216.9165625403198021 ) ) ;
#11726=CARTESIAN_POINT ( 'NONE',  ( -47.82626200431142394, -294.3859196442186317, -342.8188357746217889 ) ) ;
#11728=CARTESIAN_POINT ( 'NONE',  ( -98.95245104799202807, -289.2875037354023675, -316.3984167867946553 ) ) ;
#11729=CARTESIAN_POINT ( 'NONE',  ( 16.72988289493238057, -285.0747629120200486, -219.8029399253381371 ) ) ;
#11730=CARTESIAN_POINT ( 'NONE',  ( -5.527607383993497159, -285.0537078233779766, -203.9903196028090804 ) ) ;
#11731=CARTESIAN_POINT ( 'NONE',  ( -109.3413263621045672, -288.5688874194672167, -287.5083579527609459 ) ) ;
#11732=CARTESIAN_POINT ( 'NONE',  ( -107.3600760673499366, -285.4670424617925164, -292.3737856042744170 ) ) ;
#11733=CARTESIAN_POINT ( 'NONE',  ( 9.262817734426024074, -274.4122399569943695, -329.1898158302455499 ) ) ;
#11734=CARTESIAN_POINT ( 'NONE',  ( -23.90671828721737668, -284.6207606491204842, -195.3011844166014725 ) ) ;
#11735=CARTESIAN_POINT ( 'NONE',  ( -48.69310354446782441, -299.9079007241820705, -196.1728451924504952 ) ) ;
#11736=CARTESIAN_POINT ( 'NONE',  ( 17.29431629925166547, -286.2742332370357303, -321.9841180463167234 ) ) ;
#11737=CARTESIAN_POINT ( 'NONE',  ( -9.167869994485087659, -281.3710761509059353, -202.7619778689879979 ) ) ;
#11738=CARTESIAN_POINT ( 'NONE',  ( -56.79135804319869152, -291.3023910024834322, -343.0216492172917242 ) ) ;
#11741=CARTESIAN_POINT ( 'NONE',  ( -27.90300671838431157, -296.8534991211220699, -345.3815764387252898 ) ) ;
#11742=CARTESIAN_POINT ( 'NONE',  ( -80.17683077337308362, -277.4719795954232495, -208.7969057410843163 ) ) ;
#11743=CARTESIAN_POINT ( 'NONE',  ( -72.09007957810054279, -290.8016131279472916, -201.8140108161004207 ) ) ;
#11744=CARTESIAN_POINT ( 'NONE',  ( -96.73212947363174408, -295.5596340879585568, -226.5309178835082378 ) ) ;
#11745=CARTESIAN_POINT ( 'NONE',  ( 16.17354225024463688, -280.9580061116063234, -320.8067575354481846 ) ) ;
#11746=CARTESIAN_POINT ( 'NONE',  ( -21.60625329655805871, -272.3352913046833805, -197.6032324449385271 ) ) ;
#11747=CARTESIAN_POINT ( 'NONE',  ( 17.45939652356535987, -295.5632921491301204, -319.3503253922410181 ) ) ;
#11748=CARTESIAN_POINT ( 'NONE',  ( 31.98288692825981272, -290.4805209788416391, -303.7098442033570223 ) ) ;
#11749=CARTESIAN_POINT ( 'NONE',  ( -62.59715637206504368, -296.2092224565062679, -198.3550787787695526 ) ) ;
#11750=CARTESIAN_POINT ( 'NONE',  ( 37.85251465581007579, -291.6488165154114540, -259.0618612532959446 ) ) ;
#11751=CARTESIAN_POINT ( 'NONE',  ( -102.1535652485686256, -291.5046454847147857, -305.3230467993019488 ) ) ;
#11753=CARTESIAN_POINT ( 'NONE',  ( -65.39831883214733921, -292.4786069832919679, -202.7796229373281562 ) ) ;
#11755=CARTESIAN_POINT ( 'NONE',  ( -30.39222680375099372, -280.9847636096063184, -345.3951877304016875 ) ) ;
#11756=CARTESIAN_POINT ( 'NONE',  ( -34.85728298530064251, -292.0842281890849677, -197.4034064541639566 ) ) ;
#11757=CARTESIAN_POINT ( 'NONE',  ( 39.27810925450119584, -281.6541718384929140, -278.5185280903869511 ) ) ;
#11758=CARTESIAN_POINT ( 'NONE',  ( -65.24848116184352875, -283.0737654950311253, -342.1176060608789271 ) ) ;
#11759=CARTESIAN_POINT ( 'NONE',  ( -26.22713541370747592, -286.9103189059982810, -344.4167914571044662 ) ) ;
#11760=CARTESIAN_POINT ( 'NONE',  ( -48.53796866150762668, -281.3357794512028249, -343.7471455981579425 ) ) ;
#11761=CARTESIAN_POINT ( 'NONE',  ( -48.00259242569042328, -278.3989126251840958, -194.7494835698466602 ) ) ;
#11762=CARTESIAN_POINT ( 'NONE',  ( 30.08434164730011062, -286.9483550530452476, -307.0128268430932508 ) ) ;
#11764=CARTESIAN_POINT ( 'NONE',  ( 23.23304758720301422, -294.5707959261951601, -228.1827175810766732 ) ) ;
#11765=CARTESIAN_POINT ( 'NONE',  ( -31.47723787421008979, -278.4048796134323993, -346.5987331437362968 ) ) ;
#11766=CARTESIAN_POINT ( 'NONE',  ( -71.66787631362498701, -277.1855977076144200, -334.8252113265434105 ) ) ;
#11767=CARTESIAN_POINT ( 'NONE',  ( -27.85119685655844535, -292.3360322400757809, -193.8945498252629420 ) ) ;
#11768=CARTESIAN_POINT ( 'NONE',  ( -80.75458304236330775, -281.7155013947428870, -332.2684242999184221 ) ) ;
#11769=CARTESIAN_POINT ( 'NONE',  ( 33.53894712342368223, -292.3684801669259059, -251.9398722610837069 ) ) ;
#11770=CARTESIAN_POINT ( 'NONE',  ( -100.6150815138749977, -295.0938930828261277, -230.0935149264976758 ) ) ;
#11773=CARTESIAN_POINT ( 'NONE',  ( 10.32693495289770702, -293.8807372098407313, -325.7297884649692605 ) ) ;
#11774=FACE_BOUND ( 'NONE', #56566, .T. ) ;
#11775=CARTESIAN_POINT ( 'NONE',  ( -92.05005921254146983, -288.6952119285918457, -226.6919474004047572 ) ) ;
#11776=CARTESIAN_POINT ( 'NONE',  ( -36.88651872117245034, -297.1164735630179621, -193.5964809375084030 ) ) ;
#11777=CARTESIAN_POINT ( 'NONE',  ( 35.99021109349600067, -279.9340052404979247, -289.4067547463413916 ) ) ;
#11780=CARTESIAN_POINT ( 'NONE',  ( 15.94364210691151484, -288.1037122962427475, -215.4614770469405300 ) ) ;
#11781=CARTESIAN_POINT ( 'NONE',  ( -84.68664261970612017, -289.5590650814730793, -325.9927252284525139 ) ) ;
#11782=CARTESIAN_POINT ( 'NONE',  ( -108.8400967152963403, -279.8382973938271334, -288.2648901868055873 ) ) ;
#11783=CARTESIAN_POINT ( 'NONE',  ( -78.88563823001278763, -293.6348069637433014, -332.4392710130770752 ) ) ;
#11784=CARTESIAN_POINT ( 'NONE',  ( -41.95356932101942959, -299.7533800294712591, -196.4916068367509183 ) ) ;
#11785=CARTESIAN_POINT ( 'NONE',  ( -110.7893362632360805, -277.3436170816679578, -270.6242444570373209 ) ) ;
#11787=CARTESIAN_POINT ( 'NONE',  ( -113.8624312931764138, -272.4927491730388738, -261.7833731474086676 ) ) ;
#11788=CARTESIAN_POINT ( 'NONE',  ( -48.24827296263730148, -291.1120298774809498, -344.0498264543599021 ) ) ;
#11789=CARTESIAN_POINT ( 'NONE',  ( 38.05723960318069743, -295.0085439118863064, -258.9877242958766033 ) ) ;
#11790=CARTESIAN_POINT ( 'NONE',  ( 201.6516428717762608, 292.4574023500951512, -53.99999999997706368 ) ) ;
#11791=CARTESIAN_POINT ( 'NONE',  ( -108.7605268715318374, -290.9974035083213835, -286.0155553866644027 ) ) ;
#11794=CARTESIAN_POINT ( 'NONE',  ( -91.56952993098747129, -297.9554750583028522, -215.8390558306278706 ) ) ;
#11795=CARTESIAN_POINT ( 'NONE',  ( -110.4347962095075104, -288.9461554691451397, -250.3694094784423214 ) ) ;
#11796=CARTESIAN_POINT ( 'NONE',  ( -89.59706575995504352, -297.6729351026829704, -213.7635042708118931 ) ) ;
#11798=FACE_OUTER_BOUND ( 'NONE', #16591, .T. ) ;
#11799=CARTESIAN_POINT ( 'NONE',  ( 5.187096875363059745, -290.0083104836809866, -333.7173266510132521 ) ) ;
#11800=CARTESIAN_POINT ( 'NONE',  ( -2.659677404128715672, -282.9805209788415823, -198.2697987213421698 ) ) ;
#11801=CARTESIAN_POINT ( 'NONE',  ( -111.4308302195787661, -286.6877879847500026, -259.8335717846267130 ) ) ;
#11802=CARTESIAN_POINT ( 'NONE',  ( 33.32150121606481008, -285.7530049581886260, -241.1484515462541367 ) ) ;
#11803=CARTESIAN_POINT ( 'NONE',  ( -18.79317459280651548, -272.2912262461288719, -197.8092274115205953 ) ) ;
#11804=CARTESIAN_POINT ( 'NONE',  ( -93.11293265455064727, -275.1630468386803159, -221.0571240069463101 ) ) ;
#11805=CARTESIAN_POINT ( 'NONE',  ( -110.6003346563089877, -288.4611142822752186, -283.5704581172514054 ) ) ;
#11806=CARTESIAN_POINT ( 'NONE',  ( -34.31631551368566591, -278.8749037063864762, -346.0654938829343905 ) ) ;
#11808=CARTESIAN_POINT ( 'NONE',  ( -41.05118505629953773, -280.0041679465415996, -197.4554273845873524 ) ) ;
#11809=CARTESIAN_POINT ( 'NONE',  ( 33.55647239966744166, -280.6653617867252137, -252.4961469644773047 ) ) ;
#11810=CARTESIAN_POINT ( 'NONE',  ( 25.82015139036784745, -277.2094185429656363, -313.9510211707606118 ) ) ;
#11811=CARTESIAN_POINT ( 'NONE',  ( 22.57439089600631021, -279.7045637080174174, -222.6111188941444539 ) ) ;
#11812=CARTESIAN_POINT ( 'NONE',  ( -107.3525364133518849, -259.7561089835505186, -315.8720887335824727 ) ) ;
#11813=CARTESIAN_POINT ( 'NONE',  ( -5.223660991503157547, -275.4058667572645049, -200.6384403523648530 ) ) ;
#11815=CARTESIAN_POINT ( 'NONE',  ( -100.6443058047159553, -274.6397606081572462, -227.6584728236507829 ) ) ;
#11816=CARTESIAN_POINT ( 'NONE',  ( -37.37352853689063892, -294.5519495502701943, -195.3611179825600175 ) ) ;
#11820=CARTESIAN_POINT ( 'NONE',  ( 25.96991669313003825, -289.1381429757798855, -307.4191197812877476 ) ) ;
#11821=CARTESIAN_POINT ( 'NONE',  ( 31.95012996263987759, -289.7159460382678731, -301.5479147726393307 ) ) ;
#11822=CARTESIAN_POINT ( 'NONE',  ( -95.85489269177629978, -289.2862853594372723, -314.2009448446495981 ) ) ;
#11823=CARTESIAN_POINT ( 'NONE',  ( -65.84872774809066698, -285.1967355518366389, -198.8845636537164410 ) ) ;
#11825=CARTESIAN_POINT ( 'NONE',  ( 32.98754730838870586, -280.2473129105107432, -292.8933919597594695 ) ) ;
#11826=CARTESIAN_POINT ( 'NONE',  ( -31.75514733084627039, -290.8414603354181054, -344.4372960680524329 ) ) ;
#11827=CARTESIAN_POINT ( 'NONE',  ( -33.47906054805210374, -281.4825587910334548, -343.9658460776556126 ) ) ;
#11828=CARTESIAN_POINT ( 'NONE',  ( -108.2920067222448921, -279.6158749119506410, -289.5261244584051497 ) ) ;
#11829=CARTESIAN_POINT ( 'NONE',  ( -80.85100677912684830, -278.1533820175014853, -329.0546327539217373 ) ) ;
#11830=CARTESIAN_POINT ( 'NONE',  ( -112.7783104193172363, -289.5144841047574005, -257.0447165564938246 ) ) ;
#11831=CARTESIAN_POINT ( 'NONE',  ( -112.9761822890654912, -285.1815137696266902, -284.2023576766145538 ) ) ;
#11832=CARTESIAN_POINT ( 'NONE',  ( 27.08280086380950991, -287.4914927807429876, -228.3015105766904469 ) ) ;
#11833=CARTESIAN_POINT ( 'NONE',  ( 20.18228246193993414, -282.3523327063134616, -315.3054327678537447 ) ) ;
#11836=CARTESIAN_POINT ( 'NONE',  ( -83.53236201604286748, -293.2871538132972660, -210.2389378926997665 ) ) ;
#11837=CARTESIAN_POINT ( 'NONE',  ( -79.30981323136398942, -290.1836321062335742, -206.3292459575291957 ) ) ;
#11838=CARTESIAN_POINT ( 'NONE',  ( 5.323522573438709493, -273.7038557481634484, -210.7745949941079573 ) ) ;
#11839=CARTESIAN_POINT ( 'NONE',  ( -34.86624419779202810, -294.3704082286992048, -347.2193309779238461 ) ) ;
#11840=CARTESIAN_POINT ( 'NONE',  ( -41.61385774977839702, -290.4773847918907563, -196.7413988045967699 ) ) ;
#11841=CARTESIAN_POINT ( 'NONE',  ( -93.87066067648564172, -294.1221814493834472, -318.1557593804848807 ) ) ;
#11842=B_SPLINE_CURVE_WITH_KNOTS ( 'NONE', 3,
 ( #49946, #37144, #86865, #58473, #22019, #65596, #1164, #64211, #30047, #87317, #14913, #22465, #85473, #20620, #21075, #42846, #49491, #71762, #8713, #10576, #81155, #2565, #81611, #30503, #51798, #66501, #59874, #74051 ),
 .UNSPECIFIED., .F., .F.,
 ( 4, 2, 2, 2, 2, 2, 2, 2, 2, 2, 2, 2, 2, 4 ),
 ( 0.006505935382142305663, 0.006896669962658084560, 0.007287404543173863457, 0.007678139123689642354, 0.008068873704205420383, 0.008459608284721200147, 0.008850342865236978177, 0.009241077445752757941, 0.009631812026268535970, 0.01041328118730009203, 0.01119475034833164982, 0.01158548492884745734, 0.01197621950936326660, 0.01275768867039482266 ),
 .UNSPECIFIED. ) ;
#11843=CARTESIAN_POINT ( 'NONE',  ( -63.95061020473567481, -290.6120151509840639, -338.8195136740945941 ) ) ;
#11845=CARTESIAN_POINT ( 'NONE',  ( -111.1601629958731507, -292.3811216796044050, -283.6938090988346062 ) ) ;
#11846=CARTESIAN_POINT ( 'NONE',  ( -1.651351009163778416, -290.5239215389173637, -204.2080575212583256 ) ) ;
#11847=CARTESIAN_POINT ( 'NONE',  ( 34.93054123707709380, -295.8122833016357163, -290.5912999540839792 ) ) ;
#11848=CARTESIAN_POINT ( 'NONE',  ( -17.11836718601185936, -287.2608417565090804, -199.9204242047243554 ) ) ;
#11849=CARTESIAN_POINT ( 'NONE',  ( -9.053773662506463538, -296.6833939349633624, -340.0569250178330094 ) ) ;
#11850=CARTESIAN_POINT ( 'NONE',  ( 37.11466220994713439, -277.6845312497366649, -282.2934803350398170 ) ) ;
#11851=CARTESIAN_POINT ( 'NONE',  ( 21.41613360024045321, -275.0119424398041019, -319.5091158610763955 ) ) ;
#11853=CARTESIAN_POINT ( 'NONE',  ( -98.95681923200736207, -296.3614924859028861, -224.4290767416403583 ) ) ;
#11854=CARTESIAN_POINT ( 'NONE',  ( -48.78634528543979343, -275.4396036881377086, -343.5363659927569415 ) ) ;
#11855=CARTESIAN_POINT ( 'NONE',  ( -71.58269891887039194, -277.6760637381186143, -204.2493401320581654 ) ) ;
#11856=CARTESIAN_POINT ( 'NONE',  ( -106.6865357460839334, -274.0753466474948254, -246.3106652291610033 ) ) ;
#11857=CARTESIAN_POINT ( 'NONE',  ( -21.45941477323787794, -272.8267042362189727, -195.6191665549959566 ) ) ;
#11858=CARTESIAN_POINT ( 'NONE',  ( -101.9762590594997675, -297.5010479940899017, -305.5427709767504325 ) ) ;
#11860=CARTESIAN_POINT ( 'NONE',  ( -66.89392010452345971, -298.4575382553139775, -203.4200729694276504 ) ) ;
#11862=CARTESIAN_POINT ( 'NONE',  ( -74.86696263462846446, -287.5693706703454495, -335.7083556989466615 ) ) ;
#11863=CARTESIAN_POINT ( 'NONE',  ( -74.27155067695211699, -273.3801315311856115, -207.3328386040565761 ) ) ;
#11864=CARTESIAN_POINT ( 'NONE',  ( 22.09017432804451531, -286.8943748884699971, -221.4034597600582401 ) ) ;
#11865=CARTESIAN_POINT ( 'NONE',  ( -4.345976336065635159, -288.2958086325601812, -339.9243277616816385 ) ) ;
#11866=CARTESIAN_POINT ( 'NONE',  ( -109.2513031221235451, -298.8232467559110432, -247.6620655784195435 ) ) ;
#11867=CARTESIAN_POINT ( 'NONE',  ( -38.39297099805281022, -293.0652040566474739, -345.1870711011701474 ) ) ;
#11868=CARTESIAN_POINT ( 'NONE',  ( 22.39126835378041847, -281.3990173969403941, -318.7154159960040829 ) ) ;
#11871=CARTESIAN_POINT ( 'NONE',  ( -111.5124260985978992, -276.6958976484647224, -259.1533272852826713 ) ) ;
#11873=CARTESIAN_POINT ( 'NONE',  ( -66.50082156175574255, -288.2375346325468968, -337.7717712545001518 ) ) ;
#11876=CARTESIAN_POINT ( 'NONE',  ( -75.76173359790544737, -287.5647585581627936, -334.7881783211586253 ) ) ;
#11877=CARTESIAN_POINT ( 'NONE',  ( -52.82257436235986603, -299.4507331487625379, -198.1506198083567654 ) ) ;
#11878=CARTESIAN_POINT ( 'NONE',  ( 37.84903145169399608, -283.1497351497974932, -284.0338941800599173 ) ) ;
#11879=CARTESIAN_POINT ( 'NONE',  ( -36.88335263032297462, -296.0779758395780163, -195.0060632432097236 ) ) ;
#11880=CARTESIAN_POINT ( 'NONE',  ( -106.1737312355437126, -284.2267880142716763, -294.8252525044101731 ) ) ;
#11881=CARTESIAN_POINT ( 'NONE',  ( -62.24603790994116537, -275.1470580657255596, -201.1141044985861015 ) ) ;
#11882=CARTESIAN_POINT ( 'NONE',  ( -36.79343992032838884, -282.0592019801688366, -195.3504113958989876 ) ) ;
#11884=CARTESIAN_POINT ( 'NONE',  ( -55.33992824315551928, -296.8737459230746367, -199.3194009591837528 ) ) ;
#11885=ORIENTED_EDGE ( 'NONE', *, *, #2379, .T. ) ;
#11887=CARTESIAN_POINT ( 'NONE',  ( -13.78406194055809664, -294.5879634934768774, -343.6689462652067846 ) ) ;
#11888=CARTESIAN_POINT ( 'NONE',  ( -109.6276565220233579, -286.7723836883359354, -251.7442623429170681 ) ) ;
#11890=CARTESIAN_POINT ( 'NONE',  ( -2.659677404128736544, -280.1237833571632336, -342.4524372437778652 ) ) ;
#11891=CARTESIAN_POINT ( 'NONE',  ( -41.38619084396332681, -276.2990005151955302, -347.1063061983342095 ) ) ;
#11893=CARTESIAN_POINT ( 'NONE',  ( -110.7765126455665978, -288.6945117161553753, -290.7024239173342721 ) ) ;
#11894=CARTESIAN_POINT ( 'NONE',  ( 12.39879054353536958, -283.8642601007659323, -324.7356647737787512 ) ) ;
#11895=CARTESIAN_POINT ( 'NONE',  ( -13.43720181756111565, -278.4977468912605900, -340.4617628390448658 ) ) ;
#11896=CARTESIAN_POINT ( 'NONE',  ( -31.66183847170702492, -284.4070772694444145, -346.5736641192407888 ) ) ;
#11897=CARTESIAN_POINT ( 'NONE',  ( -104.4826819890446075, -282.9501992718563770, -300.0127462419482640 ) ) ;
#11898=CARTESIAN_POINT ( 'NONE',  ( -80.21855741976330023, -281.4716564336793567, -208.8259592917643204 ) ) ;
#11899=CARTESIAN_POINT ( 'NONE',  ( -15.77939409296619289, -274.4901564271136749, -196.3864521335050313 ) ) ;
#11900=CARTESIAN_POINT ( 'NONE',  ( -69.01731485000155430, -277.2906191478002143, -340.5585366834978345 ) ) ;
#11901=CARTESIAN_POINT ( 'NONE',  ( -66.59698157317149025, -297.3585213228496968, -338.8114116806738707 ) ) ;
#11904=CARTESIAN_POINT ( 'NONE',  ( -92.80172060689096725, -293.9765023789503289, -321.9989462706197969 ) ) ;
#11905=CARTESIAN_POINT ( 'NONE',  ( -1.445459428485909248, -276.0704572094677474, -334.0536412462648741 ) ) ;
#11906=CARTESIAN_POINT ( 'NONE',  ( -36.55841889359908237, -299.1414084624087195, -193.6700876241062872 ) ) ;
#11907=CARTESIAN_POINT ( 'NONE',  ( -7.871784015579938121, -288.2038361082733786, -202.4678336343174578 ) ) ;
#11908=CARTESIAN_POINT ( 'NONE',  ( 37.08075170875183346, -294.8589223784181286, -253.4501109912460493 ) ) ;
#11909=CARTESIAN_POINT ( 'NONE',  ( 31.87783838519173685, -295.1812889064271417, -303.2973836299144637 ) ) ;
#11910=CARTESIAN_POINT ( 'NONE',  ( -105.7126183004163664, -292.1513018800488908, -300.9101353951804754 ) ) ;
#11911=CARTESIAN_POINT ( 'NONE',  ( -46.66011258465849210, -277.9335628587383553, -196.0578377145540969 ) ) ;
#11912=CARTESIAN_POINT ( 'NONE',  ( -97.58519442977799940, -281.0723888527524537, -226.6342887573707969 ) ) ;
#11913=CARTESIAN_POINT ( 'NONE',  ( -101.4182199183619133, -294.1202938809319676, -308.3508446733941923 ) ) ;
#11914=CARTESIAN_POINT ( 'NONE',  ( 6.234265778095955390, -284.3283624284052280, -332.4046432469247065 ) ) ;
#11915=CARTESIAN_POINT ( 'NONE',  ( -8.119147141539352575, -285.3644825102141453, -203.1281761218491511 ) ) ;
#11916=CARTESIAN_POINT ( 'NONE',  ( -75.84180017535200591, -209.4652300186797049, -356.3057796646524480 ) ) ;
#11917=VERTEX_POINT ( 'NONE', #16764 ) ;
#11918=CARTESIAN_POINT ( 'NONE',  ( -97.37090427723909158, -284.7982187592184005, -228.7627968174912496 ) ) ;
#11920=CARTESIAN_POINT ( 'NONE',  ( 4.389075172492190369, -283.5835164434987519, -334.7669925542786018 ) ) ;
#11921=CARTESIAN_POINT ( 'NONE',  ( -59.48609328469245838, -274.0907847944768037, -200.7257587572469788 ) ) ;
#11922=CARTESIAN_POINT ( 'NONE',  ( -63.05363600282146308, -284.5195216888135405, -198.2022302990849880 ) ) ;
#11923=CARTESIAN_POINT ( 'NONE',  ( 29.07698386091632514, -281.9913298667300978, -231.8724361448573745 ) ) ;
#11925=CARTESIAN_POINT ( 'NONE',  ( -31.14950356325812564, -281.6490172806020382, -194.2538922277914537 ) ) ;
#11926=CARTESIAN_POINT ( 'NONE',  ( -1.190700509482957470, -281.1704389952192287, -202.4905204206547751 ) ) ;
#11927=CARTESIAN_POINT ( 'NONE',  ( -37.37352853689063181, -286.5523547857346784, -340.3611179825599606 ) ) ;
#11928=CARTESIAN_POINT ( 'NONE',  ( -38.73072492404651257, -140.1446639439760702, -364.8181740665336292 ) ) ;
#11930=CARTESIAN_POINT ( 'NONE',  ( -67.82711616010269040, -275.6512994770065461, -202.0047941750336520 ) ) ;
#11931=CARTESIAN_POINT ( 'NONE',  ( -31.67332922037059006, -124.0639957142015533, -364.0958594919561051 ) ) ;
#11932=CARTESIAN_POINT ( 'NONE',  ( -105.9440327837278915, -276.9587884342035977, -240.9406021121017147 ) ) ;
#11933=CARTESIAN_POINT ( 'NONE',  ( -37.81155663608277706, -293.8064773571610999, -194.3759006540348935 ) ) ;
#11934=CARTESIAN_POINT ( 'NONE',  ( -97.27169148441737434, -295.3178765231755278, -312.2214668146835379 ) ) ;
#11935=CARTESIAN_POINT ( 'NONE',  ( -90.73871056436745164, -290.8272698274044501, -214.8950699995339733 ) ) ;
#11937=CARTESIAN_POINT ( 'NONE',  ( -106.6396837845702237, -294.7116974572602430, -302.5542189893770342 ) ) ;
#11938=CARTESIAN_POINT ( 'NONE',  ( 32.60525647443726882, -285.6427788552146581, -246.8268094768048115 ) ) ;
#11939=CARTESIAN_POINT ( 'NONE',  ( 22.79158483978172356, -294.8134448020422269, -226.8095953903694806 ) ) ;
#11940=CARTESIAN_POINT ( 'NONE',  ( 33.55319126898695714, -286.4933798103258482, -289.9187965230924533 ) ) ;
#11941=CARTESIAN_POINT ( 'NONE',  ( -92.92116950648502893, -285.1865728186486990, -318.4652515098845811 ) ) ;
#11943=CARTESIAN_POINT ( 'NONE',  ( -50.53772762970902477, -292.8288226814275390, -194.7391299729637808 ) ) ;
#11944=CARTESIAN_POINT ( 'NONE',  ( 13.97236240340401814, -282.8008410370684942, -322.4405811189353130 ) ) ;
#11945=CARTESIAN_POINT ( 'NONE',  ( -102.7843733399455743, -294.8245010074130619, -310.1765074795446822 ) ) ;
#11946=CARTESIAN_POINT ( 'NONE',  ( -82.74897544549313011, -290.4583979378410845, -332.3477146650190548 ) ) ;
#11947=CARTESIAN_POINT ( 'NONE',  ( -11.18007883237300604, -292.8763495210278052, -197.9511605447531508 ) ) ;
#11948=CARTESIAN_POINT ( 'NONE',  ( 33.38803480352928688, -287.4797993331431485, -252.2467664456233933 ) ) ;
#11951=CARTESIAN_POINT ( 'NONE',  ( -96.42900093387635252, -297.7665343754947003, -317.8052274613804684 ) ) ;
#11952=CARTESIAN_POINT ( 'NONE',  ( -84.89671618182417490, -296.0964742166052588, -210.4293340983272742 ) ) ;
#11953=CARTESIAN_POINT ( 'NONE',  ( 27.99671797459161482, -280.1618587805434117, -237.1684379888619674 ) ) ;
#11955=CARTESIAN_POINT ( 'NONE',  ( 35.14088228149329041, -275.3874989983887076, -296.3212588594157637 ) ) ;
#11957=CARTESIAN_POINT ( 'NONE',  ( -110.9032408041161091, -295.0895906233503183, -265.9557253485581327 ) ) ;
#11958=CARTESIAN_POINT ( 'NONE',  ( -51.49354218856608156, -279.0954822059095477, -343.2349187883628474 ) ) ;
#11959=CARTESIAN_POINT ( 'NONE',  ( -27.09665949279046160, -272.3231992950544509, -196.7844998258825342 ) ) ;
#11960=CARTESIAN_POINT ( 'NONE',  ( -18.10171823212836273, -296.0036361283404176, -341.1915747111040673 ) ) ;
#11961=CARTESIAN_POINT ( 'NONE',  ( -63.20132276407057503, -298.7870346821795238, -201.7107164865911102 ) ) ;
#11963=CARTESIAN_POINT ( 'NONE',  ( -48.86929473770263144, -299.5079330296687203, -194.9850034571304320 ) ) ;
#11964=CARTESIAN_POINT ( 'NONE',  ( -56.88783298730761118, -295.8006349718829142, -197.7263289338401933 ) ) ;
#11965=CARTESIAN_POINT ( 'NONE',  ( -28.10167507329012437, -292.8238083442508355, -197.7946828861999791 ) ) ;
#11966=CARTESIAN_POINT ( 'NONE',  ( -94.73917262081765500, -289.7727667268370624, -224.2878146096032594 ) ) ;
#11968=CARTESIAN_POINT ( 'NONE',  ( -0.08074427398172294434, -275.0265562188263289, -203.0323343567650909 ) ) ;
#11969=CARTESIAN_POINT ( 'NONE',  ( -103.2059893864593931, -273.1445513411402430, -238.8826268342931201 ) ) ;
#11970=CARTESIAN_POINT ( 'NONE',  ( 9.774517450236274385, -282.6765479314079812, -211.4855070770204577 ) ) ;
#11971=CARTESIAN_POINT ( 'NONE',  ( -52.83422942530944511, -281.9313824124492385, -345.3370881873298686 ) ) ;
#11972=CARTESIAN_POINT ( 'NONE',  ( -2.778368391850212671, -275.9559438820924129, -339.0684893653298104 ) ) ;
#11973=CARTESIAN_POINT ( 'NONE',  ( -103.1623985106912613, -283.3164742530137232, -302.4186551696149081 ) ) ;
#11974=CARTESIAN_POINT ( 'NONE',  ( 37.58628065862232148, -279.4753064740824016, -264.3756255478745061 ) ) ;
#11975=CARTESIAN_POINT ( 'NONE',  ( -93.35054011315504852, -271.8005968509393711, -222.6092437142021367 ) ) ;
#11976=CARTESIAN_POINT ( 'NONE',  ( -112.2711749018781546, -280.6072150155323470, -266.0855091339631144 ) ) ;
#11979=CARTESIAN_POINT ( 'NONE',  ( -67.75106180120246790, -295.8985455865802123, -200.6685581360634103 ) ) ;
#11980=CARTESIAN_POINT ( 'NONE',  ( 30.21892019334217849, -277.9870224707883040, -303.4280633812549581 ) ) ;
#11981=CARTESIAN_POINT ( 'NONE',  ( 20.55867556936468077, -272.8944578681928874, -222.6898777343884888 ) ) ;
#11983=CARTESIAN_POINT ( 'NONE',  ( -110.8131001222128162, -286.2467500528933897, -288.0585939169493486 ) ) ;
#11986=CARTESIAN_POINT ( 'NONE',  ( 6.047021010661475238, -286.4638105083834034, -331.5991299858230263 ) ) ;
#11988=CARTESIAN_POINT ( 'NONE',  ( -0.5722527155605370286, -293.3471525912123639, -333.9418572773470260 ) ) ;
#11989=CARTESIAN_POINT ( 'NONE',  ( 22.95130391865977515, -286.2871191324499591, -313.6695368501304984 ) ) ;
#11990=CARTESIAN_POINT ( 'NONE',  ( -82.08396892746139883, -205.6231916066184624, -355.0661004095303497 ) ) ;
#11991=CARTESIAN_POINT ( 'NONE',  ( -96.36268795855517055, -293.9168872256790905, -316.6377173474196525 ) ) ;
#11992=CARTESIAN_POINT ( 'NONE',  ( -97.02588882726561792, -283.6743962815139071, -222.8163456593140666 ) ) ;
#11993=CARTESIAN_POINT ( 'NONE',  ( 9.771765009306662364, -282.3131028808741121, -213.4899239032754394 ) ) ;
#11994=CARTESIAN_POINT ( 'NONE',  ( -3.677768561452260165, -287.6915676875727286, -201.5371584017965461 ) ) ;
#11995=CARTESIAN_POINT ( 'NONE',  ( 37.42443782884210890, -279.9648363296811340, -283.9978842131654915 ) ) ;
#11996=CARTESIAN_POINT ( 'NONE',  ( -34.57800184039527380, -289.0166003900959026, -343.3583656645191695 ) ) ;
#11997=CARTESIAN_POINT ( 'NONE',  ( -22.08986493811561047, -281.6765148138701989, -198.3174808447351722 ) ) ;
#11998=CARTESIAN_POINT ( 'NONE',  ( -3.082510429314294420, -281.3197669460260499, -205.7024231446197859 ) ) ;
#12000=CARTESIAN_POINT ( 'NONE',  ( 35.10280011080594420, -289.2642166040210441, -249.4347683480205831 ) ) ;
#12002=CARTESIAN_POINT ( 'NONE',  ( -113.8626674886053678, -272.6594023460276617, -261.7854807345403856 ) ) ;
#12003=CARTESIAN_POINT ( 'NONE',  ( -74.33876776348557769, -291.5264750778824805, -335.2068920707291113 ) ) ;
#12005=CARTESIAN_POINT ( 'NONE',  ( -69.91165696735023971, -276.1233781216988064, -202.8022627189028810 ) ) ;
#12007=CARTESIAN_POINT ( 'NONE',  ( -20.56077931937331726, -274.8371346808540352, -343.6840942699477637 ) ) ;
#12009=CARTESIAN_POINT ( 'NONE',  ( -61.35894570803728243, -293.7587048365227247, -342.7323422057019116 ) ) ;
#12010=CARTESIAN_POINT ( 'NONE',  ( -93.65699342930312810, -296.7193012729372867, -223.7951624828971546 ) ) ;
#12011=CARTESIAN_POINT ( 'NONE',  ( -39.96340923975267856, -290.6056837565198521, -344.0578511618480206 ) ) ;
#12012=CARTESIAN_POINT ( 'NONE',  ( 8.438090839920427300, -284.1760635549513836, -328.5831412016553372 ) ) ;
#12013=CARTESIAN_POINT ( 'NONE',  ( -108.2449011334998090, -291.6131318147539560, -298.8451903521631721 ) ) ;
#12014=CARTESIAN_POINT ( 'NONE',  ( -111.0622698857904993, -291.6093430813161262, -290.8202447521590557 ) ) ;
#12015=CARTESIAN_POINT ( 'NONE',  ( -3.720211904967436922, -288.4959754508652736, -203.3193684354497748 ) ) ;
#12016=CARTESIAN_POINT ( 'NONE',  ( -73.76751629861605863, -279.7489066921709195, -202.5069459657786695 ) ) ;
#12017=CARTESIAN_POINT ( 'NONE',  ( -109.4333787901076533, -294.3417296020811023, -293.0341870494128216 ) ) ;
#12018=CARTESIAN_POINT ( 'NONE',  ( -52.91968858602928805, -283.0796915706076788, -345.8233438824149175 ) ) ;
#12019=CARTESIAN_POINT ( 'NONE',  ( 33.70532038733049518, -277.6933128490790068, -291.9269958120816568 ) ) ;
#12021=CARTESIAN_POINT ( 'NONE',  ( -107.3452863284742449, -275.1604526064901393, -262.5058405983616012 ) ) ;
#12023=CARTESIAN_POINT ( 'NONE',  ( 29.07289954989624192, -273.3058408325565551, -233.3330177788781725 ) ) ;
#12025=CARTESIAN_POINT ( 'NONE',  ( -5.526034681492270728, -279.9900228883731756, -204.5906696483962151 ) ) ;
#12026=CARTESIAN_POINT ( 'NONE',  ( -97.60697025100625979, -279.1217732958113515, -317.6485998084235689 ) ) ;
#12028=CARTESIAN_POINT ( 'NONE',  ( -54.89911711056387134, -284.8904909920424302, -195.6312222166651509 ) ) ;
#12029=CARTESIAN_POINT ( 'NONE',  ( -17.17776363783582738, -294.0760283630731351, -199.0941106353228065 ) ) ;
#12030=CARTESIAN_POINT ( 'NONE',  ( 22.12114468027513681, -276.5070288106356884, -222.6895104939444252 ) ) ;
#12031=CARTESIAN_POINT ( 'NONE',  ( -24.26050937830338938, -275.5308541059839627, -194.9270596098099020 ) ) ;
#12033=CARTESIAN_POINT ( 'NONE',  ( 23.98323269371284638, -275.9348189188465312, -310.0554889903755225 ) ) ;
#12034=CARTESIAN_POINT ( 'NONE',  ( -110.6763679830202989, -298.3597315934669609, -285.3263355785745716 ) ) ;
#12035=CARTESIAN_POINT ( 'NONE',  ( -37.25377280838804239, -284.0530614498246109, -195.5150814858104980 ) ) ;
#12036=CARTESIAN_POINT ( 'NONE',  ( 1.693041237821428568, -292.2255401779535191, -203.9523791118493534 ) ) ;
#12037=CARTESIAN_POINT ( 'NONE',  ( 22.13250329715412335, -274.1922227026672090, -315.4683893789126614 ) ) ;
#12038=CARTESIAN_POINT ( 'NONE',  ( -7.217242680788439557, -290.2637008478211555, -340.3677651890384936 ) ) ;
#12039=CARTESIAN_POINT ( 'NONE',  ( -28.05361346976921411, -291.0930025974869864, -197.5918104978125882 ) ) ;
#12041=CARTESIAN_POINT ( 'NONE',  ( 24.34954572478147128, -291.5237045862518812, -225.2745736584487872 ) ) ;
#12042=CARTESIAN_POINT ( 'NONE',  ( -102.4264875098985783, -290.6697245900886060, -237.1424351068653209 ) ) ;
#12044=CARTESIAN_POINT ( 'NONE',  ( 32.42508598765144257, -288.2216390095728684, -238.3885792133189909 ) ) ;
#12045=CARTESIAN_POINT ( 'NONE',  ( -64.82800983640910886, -280.0162774585989496, -202.7106171313166953 ) ) ;
#12046=CARTESIAN_POINT ( 'NONE',  ( 4.048852894904261923, -293.4292338567008755, -334.9861218836370540 ) ) ;
#12047=CARTESIAN_POINT ( 'NONE',  ( -83.22171987203101651, -286.0938626919149783, -208.5829895882328913 ) ) ;
#12048=CARTESIAN_POINT ( 'NONE',  ( 35.82760768382338057, -287.5825273056528317, -246.2742231218383893 ) ) ;
#12049=CARTESIAN_POINT ( 'NONE',  ( 18.51327032795031258, -282.5535809824711464, -317.4157264960379621 ) ) ;
#12050=CARTESIAN_POINT ( 'NONE',  ( 5.697525119581973385, -58.35050878906803007, -354.7899736438976106 ) ) ;
#12051=CARTESIAN_POINT ( 'NONE',  ( -91.01950653586207807, -229.5109285105102117, -346.8848101179228252 ) ) ;
#12052=CARTESIAN_POINT ( 'NONE',  ( 187.9541643320069113, 268.7763698351266157, -137.5712847132034540 ) ) ;
#12053=CARTESIAN_POINT ( 'NONE',  ( 7.437794970279090201, -273.8781792905782595, -212.5044109801810919 ) ) ;
#12054=CARTESIAN_POINT ( 'NONE',  ( -40.53292591936764211, -276.0135128299020266, -343.6132564228390152 ) ) ;
#12055=CARTESIAN_POINT ( 'NONE',  ( -99.03933312968028702, -296.6719276773890783, -224.3725246228790127 ) ) ;
#12056=CARTESIAN_POINT ( 'NONE',  ( 180.7906440682407663, 251.0613717956916560, -164.6901867084850437 ) ) ;
#12057=CARTESIAN_POINT ( 'NONE',  ( 36.40575605637703660, -274.4942664410054363, -290.7719250130335809 ) ) ;
#12058=CARTESIAN_POINT ( 'NONE',  ( -68.73247420903742011, -275.3939662924613003, -203.3204180578236162 ) ) ;
#12060=CARTESIAN_POINT ( 'NONE',  ( -14.90765706747966490, -299.2678316286620657, -193.5929225309962476 ) ) ;
#12061=CARTESIAN_POINT ( 'NONE',  ( 28.28578510267488610, -288.4790709341182264, -302.4706434188188950 ) ) ;
#12062=CARTESIAN_POINT ( 'NONE',  ( -56.02111412153313807, -296.0896449586250583, -344.8945890734977979 ) ) ;
#12063=CARTESIAN_POINT ( 'NONE',  ( -114.3044827737108875, -297.0180482407640170, -272.4743640083499940 ) ) ;
#12064=CARTESIAN_POINT ( 'NONE',  ( 31.54075996821940109, -294.0422162593171151, -294.6828556138995054 ) ) ;
#12066=CARTESIAN_POINT ( 'NONE',  ( 21.53464059610251624, -278.1192746915972407, -317.7407597516067312 ) ) ;
#12068=CARTESIAN_POINT ( 'NONE',  ( -48.10396624039731961, -279.4265218701735307, -194.1252946922032834 ) ) ;
#12069=CARTESIAN_POINT ( 'NONE',  ( -78.75521430402318401, -278.5663156721249720, -330.8242638033912613 ) ) ;
#12070=CARTESIAN_POINT ( 'NONE',  ( 14.21235068436446625, -278.1002765565810364, -326.2552728451562984 ) ) ;
#12071=CARTESIAN_POINT ( 'NONE',  ( -111.6807755903653998, -276.4146507069258973, -282.6943520841978739 ) ) ;
#12072=CARTESIAN_POINT ( 'NONE',  ( -96.18730163186943116, -297.8108117375129495, -226.9684720651976306 ) ) ;
#12073=CARTESIAN_POINT ( 'NONE',  ( -75.98278277568226713, -294.1536051859461622, -333.0483368961862425 ) ) ;
#12075=CARTESIAN_POINT ( 'NONE',  ( -6.260979659944867493, -280.9419849285802115, -199.9656407025799467 ) ) ;
#12076=CARTESIAN_POINT ( 'NONE',  ( -93.09157462559910812, -279.3887618167108258, -223.2149169268290620 ) ) ;
#12077=CARTESIAN_POINT ( 'NONE',  ( 23.73832545172015784, -286.8544458745618044, -316.4320279948617554 ) ) ;
#12078=CARTESIAN_POINT ( 'NONE',  ( -35.89847248428284843, -300.0703343395864522, -195.1939519473317262 ) ) ;
#12080=CARTESIAN_POINT ( 'NONE',  ( -78.27320510520871721, -288.8152378342200564, -331.0621457637079175 ) ) ;
#12081=CARTESIAN_POINT ( 'NONE',  ( -11.36680714482212551, -278.6349657166464908, -201.0012190010811253 ) ) ;
#12082=CARTESIAN_POINT ( 'NONE',  ( -39.70209396986417261, -278.5966893481790976, -196.7971308432429680 ) ) ;
#12083=CARTESIAN_POINT ( 'NONE',  ( -15.73748276506246846, -280.8502940522446352, -341.5971481064415229 ) ) ;
#12085=CARTESIAN_POINT ( 'NONE',  ( 14.10028829397946737, -288.7740956177092357, -215.7133758892978790 ) ) ;
#12086=CARTESIAN_POINT ( 'NONE',  ( -92.51702009879923594, -280.4445017572029428, -221.9393641559117896 ) ) ;
#12088=CARTESIAN_POINT ( 'NONE',  ( -7.996835274825064843, -294.4366931725923564, -201.3263074816831306 ) ) ;
#12089=CARTESIAN_POINT ( 'NONE',  ( -45.56256277481169548, -275.3946948587646943, -345.9541394910341978 ) ) ;
#12090=CIRCLE ( 'NONE', #10592, 2.939656322713313230 ) ;
#12091=CARTESIAN_POINT ( 'NONE',  ( 3.197517151241683564, -277.1428203115000883, -331.1925615817715425 ) ) ;
#12092=CARTESIAN_POINT ( 'NONE',  ( -49.76481145806104678, -285.2102801587333829, -344.5466612843584358 ) ) ;
#12094=CARTESIAN_POINT ( 'NONE',  ( -88.49825579899042793, -291.6830222655178773, -325.9697594667278508 ) ) ;
#12095=CARTESIAN_POINT ( 'NONE',  ( -111.9921130698222669, -294.4525742150585188, -278.1037617474970034 ) ) ;
#12096=CARTESIAN_POINT ( 'NONE',  ( 38.62747359294239402, -286.6037749383541495, -258.7476642976691323 ) ) ;
#12098=CARTESIAN_POINT ( 'NONE',  ( -24.49386947443048967, -272.9042454923451260, -197.9477477540017105 ) ) ;
#12099=CARTESIAN_POINT ( 'NONE',  ( 34.30267206218994147, -291.9448418601630806, -289.8503127165409410 ) ) ;
#12102=CARTESIAN_POINT ( 'NONE',  ( -88.17308651892729188, -289.8354375658416870, -213.4499775204312186 ) ) ;
#12103=CARTESIAN_POINT ( 'NONE',  ( -65.41622508650461043, -287.2791818744134957, -202.0552552028171078 ) ) ;
#12104=CARTESIAN_POINT ( 'NONE',  ( 36.39894947718684648, -285.5595333313642641, -252.0228898107602618 ) ) ;
#12105=CARTESIAN_POINT ( 'NONE',  ( -107.9522164552924721, -285.7048899173073551, -291.1311737325640934 ) ) ;
#12107=CARTESIAN_POINT ( 'NONE',  ( -96.71183582797749523, -285.9517544706959029, -227.5870964547588642 ) ) ;
#12109=CARTESIAN_POINT ( 'NONE',  ( -5.326349165420787735, -294.4512190947503996, -202.1451073256325230 ) ) ;
#12110=CARTESIAN_POINT ( 'NONE',  ( 22.36485730461436816, -274.2623918198684692, -316.6902055586546680 ) ) ;
#12111=CARTESIAN_POINT ( 'NONE',  ( 39.29583067753333836, -275.7880703290786073, -262.5782603437717739 ) ) ;
#12112=CARTESIAN_POINT ( 'NONE',  ( 3.386338600675487420, -290.6744581830073457, -206.6552262671307574 ) ) ;
#12113=CARTESIAN_POINT ( 'NONE',  ( -59.30214201170247890, -279.7754927335259367, -196.5590923174327429 ) ) ;
#12114=CARTESIAN_POINT ( 'NONE',  ( -53.48097994725340243, -297.2399588052111881, -343.2934199162808113 ) ) ;
#12117=CARTESIAN_POINT ( 'NONE',  ( -67.73646410636035853, -284.3295090226798720, -203.4477276778946759 ) ) ;
#12118=CARTESIAN_POINT ( 'NONE',  ( 18.65292621928355743, -278.8573599138828740, -220.4458830727914176 ) ) ;
#12120=CARTESIAN_POINT ( 'NONE',  ( 13.51692020822867590, -273.2285297687224670, -213.4036866298212658 ) ) ;
#12121=CARTESIAN_POINT ( 'NONE',  ( -32.42197374866186976, -276.3372129110847482, -343.3473521264460828 ) ) ;
#12122=CARTESIAN_POINT ( 'NONE',  ( -47.87316328768768869, -296.7085001218731577, -343.3498152119228166 ) ) ;
#12123=CARTESIAN_POINT ( 'NONE',  ( 1.230447900359898927, -279.4745957653457822, -204.0157968305569796 ) ) ;
#12124=CARTESIAN_POINT ( 'NONE',  ( -18.14732858763413503, -295.7398548508115823, -341.0363226063383308 ) ) ;
#12125=CARTESIAN_POINT ( 'NONE',  ( -107.9136246579931964, -297.4875592714385562, -300.0430711448337320 ) ) ;
#12126=CARTESIAN_POINT ( 'NONE',  ( -104.3974404178966608, -272.6087385816778692, -241.3259865658003207 ) ) ;
#12127=CARTESIAN_POINT ( 'NONE',  ( -76.03261901806769174, -293.5358917652077366, -206.0508561117189288 ) ) ;
#12128=CARTESIAN_POINT ( 'NONE',  ( -29.46504789154979420, -286.3159943636675848, -193.7650452761536712 ) ) ;
#12129=CARTESIAN_POINT ( 'NONE',  ( 36.38432931418959271, -273.9142899411396002, -287.8748182233948114 ) ) ;
#12130=CARTESIAN_POINT ( 'NONE',  ( 35.94710223975818053, -287.6824663743896053, -293.9778800805364085 ) ) ;
#12131=CARTESIAN_POINT ( 'NONE',  ( -111.6051648534035792, -280.6356769159129954, -262.3285223940375772 ) ) ;
#12132=ADVANCED_FACE ( 'NONE', ( #44233 ), #68540, .F. ) ;
#12133=CARTESIAN_POINT ( 'NONE',  ( 35.86463821520069217, -286.6558863060381555, -273.7827368651386450 ) ) ;
#12134=CARTESIAN_POINT ( 'NONE',  ( -96.74805393107904194, -289.1794479906947117, -224.5595020958670602 ) ) ;
#12135=CARTESIAN_POINT ( 'NONE',  ( 192.3098639061998369, 281.3337059592261085, -109.1536320133224081 ) ) ;
#12136=CARTESIAN_POINT ( 'NONE',  ( 34.62912086282523916, -286.8902635349357979, -257.4982663267292651 ) ) ;
#12138=CARTESIAN_POINT ( 'NONE',  ( 21.43760079848006939, -283.1602244131310044, -319.7353419897778508 ) ) ;
#12139=CARTESIAN_POINT ( 'NONE',  ( -113.5813438005440901, -289.4929522382327036, -279.7635207484131570 ) ) ;
#12140=CARTESIAN_POINT ( 'NONE',  ( -36.77913987123995554, -281.6592347143105144, -194.1502822681547968 ) ) ;
#12141=CARTESIAN_POINT ( 'NONE',  ( 1.111525613179245697, -281.8690547907502264, -204.1596884215062460 ) ) ;
#12142=CARTESIAN_POINT ( 'NONE',  ( 0.4017681391234181332, -280.4031858349217146, -207.8171592341532516 ) ) ;
#12143=CARTESIAN_POINT ( 'NONE',  ( 20.52618475422655919, -276.8941315245025976, -222.6504425319625682 ) ) ;
#12144=CARTESIAN_POINT ( 'NONE',  ( -74.60636176672315401, -295.5334945952799330, -337.8029128380182442 ) ) ;
#12145=CARTESIAN_POINT ( 'NONE',  ( -89.05226049374094544, -289.3414026917805018, -216.4578912480474742 ) ) ;
#12146=CARTESIAN_POINT ( 'NONE',  ( 95.12591598188809883, -298.6689901460368333, -197.0771287801524352 ) ) ;
#12149=CARTESIAN_POINT ( 'NONE',  ( -85.78064239524103129, -285.6491776325273690, -326.8852992426071751 ) ) ;
#12150=CARTESIAN_POINT ( 'NONE',  ( -34.98374721744943372, -293.1607495128159826, -193.6933888333213361 ) ) ;
#12151=CARTESIAN_POINT ( 'NONE',  ( -32.13016675250568710, -283.6360914014192076, -343.2770462023576670 ) ) ;
#12152=CARTESIAN_POINT ( 'NONE',  ( -49.66960162630130782, -272.9574977029046181, -194.5391266561833561 ) ) ;
#12153=CARTESIAN_POINT ( 'NONE',  ( -113.7113057255853192, -291.0853606803837579, -279.8000047734951750 ) ) ;
#12154=CARTESIAN_POINT ( 'NONE',  ( -86.92342681083555078, -283.5107149691977497, -213.0033068358802666 ) ) ;
#12156=CARTESIAN_POINT ( 'NONE',  ( 23.08883111274378308, -293.2472353785645396, -222.6546788394745988 ) ) ;
#12157=CARTESIAN_POINT ( 'NONE',  ( 29.44611453984981964, -288.2840993630251205, -300.0073463656589183 ) ) ;
#12160=CARTESIAN_POINT ( 'NONE',  ( -105.2969866710188853, -260.2444925846916703, -315.5001506840901015 ) ) ;
#12162=CARTESIAN_POINT ( 'NONE',  ( -44.33620535657472317, -284.6590824827696338, -346.3994182778305344 ) ) ;
#12163=CARTESIAN_POINT ( 'NONE',  ( -20.19161114001082069, -289.7666405000204009, -195.3683826091709363 ) ) ;
#12165=CARTESIAN_POINT ( 'NONE',  ( 29.59109355022479804, -280.8749501981781691, -300.3893375235729764 ) ) ;
#12166=CARTESIAN_POINT ( 'NONE',  ( -14.59999215182917531, -276.4321008013143341, -343.9598331176591159 ) ) ;
#12167=CARTESIAN_POINT ( 'NONE',  ( -92.66902528389553595, -281.2570878000263974, -219.9734655407550008 ) ) ;
#12168=CARTESIAN_POINT ( 'NONE',  ( 86.42939490984008444, 81.28859003109494097, -300.3317345712586075 ) ) ;
#12169=CARTESIAN_POINT ( 'NONE',  ( 23.29091717055268873, -279.5016194973937331, -223.8392852947689846 ) ) ;
#12170=CARTESIAN_POINT ( 'NONE',  ( -100.9991269917803720, -283.0987470634276519, -231.2809142228382200 ) ) ;
#12171=CARTESIAN_POINT ( 'NONE',  ( -20.80751537109819083, -300.0165860262275714, -194.3695687811124913 ) ) ;
#12172=CARTESIAN_POINT ( 'NONE',  ( 32.68626100221049313, -293.7669239865959412, -249.3524132035507819 ) ) ;
#12174=CARTESIAN_POINT ( 'NONE',  ( -65.50052449426593171, -290.3609424753026929, -202.4628760507472123 ) ) ;
#12175=CARTESIAN_POINT ( 'NONE',  ( -7.915958199600482637, -277.3280347832439929, -341.4207115390197487 ) ) ;
#12176=CARTESIAN_POINT ( 'NONE',  ( -8.970830099267709912, -274.4337146183043501, -203.0458227968066751 ) ) ;
#12177=CARTESIAN_POINT ( 'NONE',  ( -112.1387490793718769, -271.6851727742526919, -253.4231730181333830 ) ) ;
#12178=CARTESIAN_POINT ( 'NONE',  ( -112.3417001281054723, -270.5523139186827279, -270.3356821209761165 ) ) ;
#12179=B_SPLINE_CURVE_WITH_KNOTS ( 'NONE', 3,
 ( #19649, #71267, #78367, #57529, #13506, #49929, #48518, #64194, #86374, #77418, #5930, #21525, #43307, #93026, #85910, #12557, #21062, #78826, #13971, #84972, #93487, #71745, #41407, #6873, #50403, #92076, #35745, #20121, #64659, #79309, #26765, #27230 ),
 .UNSPECIFIED., .F., .F.,
 ( 4, 2, 2, 2, 2, 2, 2, 2, 2, 2, 2, 2, 2, 2, 2, 4 ),
 ( 5.029510472558947976E-05, 0.0005389448914400213776, 0.001027594678154453330, 0.001516244464868885498, 0.002004894251583317234, 0.002982193825012181138, 0.003470843611726534810, 0.003959493398440889350, 0.004448143185155244324, 0.004936792971869597563, 0.005425442758583952536, 0.005914092545298305775, 0.006402742332012659882, 0.006891392118727013121, 0.007380041905441368094, 0.007868691692155720466 ),
 .UNSPECIFIED. ) ;
#12181=CARTESIAN_POINT ( 'NONE',  ( 34.36468109498141388, -282.4308064254109354, -255.0560012621517103 ) ) ;
#12182=CARTESIAN_POINT ( 'NONE',  ( 36.34306245447238126, -283.0769474221561381, -251.7996045828177500 ) ) ;
#12183=CARTESIAN_POINT ( 'NONE',  ( -95.84253576604854175, -284.5152067011182453, -226.5256882694470448 ) ) ;
#12184=CARTESIAN_POINT ( 'NONE',  ( 10.01386047972154358, -273.1169381897151425, -213.6912549244103161 ) ) ;
#12185=CARTESIAN_POINT ( 'NONE',  ( -3.810487204755621971, -282.3597111919590361, -204.1161606322495743 ) ) ;
#12186=CARTESIAN_POINT ( 'NONE',  ( 30.82345145232138250, -273.6586523184039379, -242.2231109509739611 ) ) ;
#12188=CARTESIAN_POINT ( 'NONE',  ( -29.97240801541454402, -275.2272902793549179, -197.4233389703065882 ) ) ;
#12190=CARTESIAN_POINT ( 'NONE',  ( -109.4581908558036076, -279.6926047155141646, -243.6863145223899778 ) ) ;
#12194=CARTESIAN_POINT ( 'NONE',  ( -107.8871901145954268, -286.7701849255651041, -242.5842992570482011 ) ) ;
#12196=CARTESIAN_POINT ( 'NONE',  ( -20.82163094983162210, -294.0319387170497407, -341.6852733604249011 ) ) ;
#12197=CARTESIAN_POINT ( 'NONE',  ( -114.2882219228515623, -289.8899927519804010, -271.2193291012045506 ) ) ;
#12198=CARTESIAN_POINT ( 'NONE',  ( 7.559225863779852617, -284.9137802728170072, -211.4585983066750146 ) ) ;
#12199=CARTESIAN_POINT ( 'NONE',  ( -46.78262172876914349, -284.5048047828813083, -197.3288132142241977 ) ) ;
#12200=CARTESIAN_POINT ( 'NONE',  ( -74.06698991887705574, -287.7870453570566838, -334.6347940558463847 ) ) ;
#12201=CARTESIAN_POINT ( 'NONE',  ( -109.5865826433986996, -285.9281213835758422, -257.3362805320824123 ) ) ;
#12202=CARTESIAN_POINT ( 'NONE',  ( 32.31697798636230345, -273.9156722045734114, -298.2979450863081752 ) ) ;
#12203=CARTESIAN_POINT ( 'NONE',  ( 37.99772346691247549, -285.8066078133404062, -258.8542976975157330 ) ) ;
#12204=CARTESIAN_POINT ( 'NONE',  ( -45.92689010823990969, -299.9434374331393087, -195.8541038121131521 ) ) ;
#12205=CARTESIAN_POINT ( 'NONE',  ( 1.808399266338743372, -284.5744438434254562, -206.1949419754272128 ) ) ;
#12206=CARTESIAN_POINT ( 'NONE',  ( -6.681819521282037044, -281.4060838330309480, -203.8389321843791606 ) ) ;
#12207=CARTESIAN_POINT ( 'NONE',  ( -94.96872272678864135, -291.8867198598726986, -318.6423902799984376 ) ) ;
#12210=CARTESIAN_POINT ( 'NONE',  ( -107.0371653761872039, -298.0924419484564396, -299.6830084152645099 ) ) ;
#12211=CARTESIAN_POINT ( 'NONE',  ( -106.2704250900716403, -276.9385234075442099, -240.8004765643772487 ) ) ;
#12212=CARTESIAN_POINT ( 'NONE',  ( 1.627045640737986965, -291.7560645211557926, -204.0764779830154225 ) ) ;
#12213=CARTESIAN_POINT ( 'NONE',  ( -111.0416378147748588, -294.9018857734444055, -274.2029402473264668 ) ) ;
#12214=CARTESIAN_POINT ( 'NONE',  ( 15.62635212349230684, -279.5056411373265632, -219.3410838375655203 ) ) ;
#12215=CARTESIAN_POINT ( 'NONE',  ( -46.32885511714368221, -272.0170786454707468, -196.4656158069768424 ) ) ;
#12216=CARTESIAN_POINT ( 'NONE',  ( 33.92837093508556023, -295.1024964109620328, -288.3004727649005190 ) ) ;
#12217=CARTESIAN_POINT ( 'NONE',  ( -110.4683760289727132, -299.2662352645559167, -253.7030783399848985 ) ) ;
#12218=CARTESIAN_POINT ( 'NONE',  ( -65.27004920581832437, -296.1737045843922829, -199.2925713611411140 ) ) ;
#12219=CARTESIAN_POINT ( 'NONE',  ( 34.52066476800799677, -292.1092301560768192, -295.2158334448697588 ) ) ;
#12220=CARTESIAN_POINT ( 'NONE',  ( -110.9260335088017513, -291.9663220036208031, -271.2101152383597764 ) ) ;
#12222=CARTESIAN_POINT ( 'NONE',  ( -107.9103373006685302, -291.6094750962571993, -251.0564767033813780 ) ) ;
#12224=CARTESIAN_POINT ( 'NONE',  ( -111.6133822124661634, -291.9936991492689344, -251.5538813231878521 ) ) ;
#12225=CARTESIAN_POINT ( 'NONE',  ( 7.586536656508338083, -278.6814628473795210, -209.7994598067362233 ) ) ;
#12226=CARTESIAN_POINT ( 'NONE',  ( 6.676241738921436131, -292.6700126829893520, -212.1252115863068184 ) ) ;
#12227=CARTESIAN_POINT ( 'NONE',  ( -31.07375881513053884, -280.1291405431306885, -193.5639622451460014 ) ) ;
#12229=CARTESIAN_POINT ( 'NONE',  ( -113.8832898643969145, -284.1163759313272976, -278.5543671618648887 ) ) ;
#12230=CARTESIAN_POINT ( 'NONE',  ( 25.77120952216590766, -286.0943649801365041, -310.5704335842223145 ) ) ;
#12231=CARTESIAN_POINT ( 'NONE',  ( -33.45484955168409158, -281.1423197847879578, -344.5072823240979005 ) ) ;
#12232=CARTESIAN_POINT ( 'NONE',  ( -74.65187693594110385, -278.0447971328082417, -203.7979265044083093 ) ) ;
#12233=CARTESIAN_POINT ( 'NONE',  ( -52.10027496992502449, -284.7879543168428427, -195.0495433521734867 ) ) ;
#12235=CARTESIAN_POINT ( 'NONE',  ( 36.08918958322248471, -295.0496659380318647, -262.4966309275322374 ) ) ;
#12236=CARTESIAN_POINT ( 'NONE',  ( -64.86575049154239991, -278.8298329513968383, -341.6983316994605389 ) ) ;
#12237=CARTESIAN_POINT ( 'NONE',  ( -110.3721857433128832, -278.2512818505545624, -267.9033186655663030 ) ) ;
#12238=CARTESIAN_POINT ( 'NONE',  ( -112.2621967214914207, -290.4958358142283146, -288.1916435425410441 ) ) ;
#12239=CARTESIAN_POINT ( 'NONE',  ( -47.09516221221688426, -281.2549789651542369, -345.2889777796481781 ) ) ;
#12240=CARTESIAN_POINT ( 'NONE',  ( 33.34065423091620772, -292.8638572597541270, -289.5767956944072807 ) ) ;
#12241=CARTESIAN_POINT ( 'NONE',  ( -97.47326855502184628, -295.1643581684585911, -225.5156464618005430 ) ) ;
#12244=CARTESIAN_POINT ( 'NONE',  ( 33.83394867336524214, -293.2778457244722290, -286.9091041001183271 ) ) ;
#12245=CARTESIAN_POINT ( 'NONE',  ( 129.8483263487583201, -299.5541904835127980, -195.3611179825600175 ) ) ;
#12246=CARTESIAN_POINT ( 'NONE',  ( 17.40634833298269157, -290.4094976428775112, -226.7417163044926838 ) ) ;
#12247=CARTESIAN_POINT ( 'NONE',  ( -112.0426122002401144, -295.8327135549497484, -252.6807913541129835 ) ) ;
#12248=CARTESIAN_POINT ( 'NONE',  ( 35.42021604417455904, -279.4220560292304185, -249.1956301611389506 ) ) ;
#12249=CARTESIAN_POINT ( 'NONE',  ( -75.87293286456544195, -286.8644720892505120, -204.2043977389613758 ) ) ;
#12250=CARTESIAN_POINT ( 'NONE',  ( 23.53523806185751610, -286.8254345529110196, -229.9831410774160645 ) ) ;
#12251=CARTESIAN_POINT ( 'NONE',  ( -95.81142191041391243, -279.4471145343522380, -315.2164341560484786 ) ) ;
#12252=CARTESIAN_POINT ( 'NONE',  ( -111.8526729088855234, -294.6298944311196237, -265.8932621870417279 ) ) ;
#12253=CARTESIAN_POINT ( 'NONE',  ( -61.32056243981657673, -297.1278680915882546, -340.4367708109081718 ) ) ;
#12255=CARTESIAN_POINT ( 'NONE',  ( -93.03791353753595672, -276.6702134207022254, -318.1634434236502216 ) ) ;
#12258=CARTESIAN_POINT ( 'NONE',  ( -110.7916707995137244, -296.5104465501717641, -247.1443520679468691 ) ) ;
#12259=CARTESIAN_POINT ( 'NONE',  ( -83.41882080653705600, -291.6096319183529317, -328.8266047662896767 ) ) ;
#12260=CARTESIAN_POINT ( 'NONE',  ( 23.40369620696903397, -295.7715792783166648, -316.3658703643342847 ) ) ;
#12261=CARTESIAN_POINT ( 'NONE',  ( 201.0264371890905295, 293.4388253988550446, -53.99999999998393463 ) ) ;
#12263=CARTESIAN_POINT ( 'NONE',  ( 32.41338023834404680, -288.4949644403909588, -292.3956429355217779 ) ) ;
#12266=CARTESIAN_POINT ( 'NONE',  ( 35.95462134410069410, -280.3234292536554904, -247.5473179570181230 ) ) ;
#12267=CARTESIAN_POINT ( 'NONE',  ( -112.5026404498714641, -297.4078133366812722, -254.0470624620327271 ) ) ;
#12268=CARTESIAN_POINT ( 'NONE',  ( -66.51754283989180294, -289.8136788822043854, -200.4391923523176615 ) ) ;
#12269=CARTESIAN_POINT ( 'NONE',  ( -98.21986154133084312, -297.5147828649090229, -223.2272780580528320 ) ) ;
#12273=CARTESIAN_POINT ( 'NONE',  ( 9.814813650075565832, -289.9367044543358247, -330.4197763981928233 ) ) ;
#12274=CARTESIAN_POINT ( 'NONE',  ( -99.86837403722181250, -294.6952119285919025, -220.4570493818173702 ) ) ;
#12275=CARTESIAN_POINT ( 'NONE',  ( 34.48932993219253973, -281.2487535259369906, -297.8131836031942044 ) ) ;
#12276=CARTESIAN_POINT ( 'NONE',  ( -82.60727683114484421, -287.4321626107948191, -210.7703805379511550 ) ) ;
#12277=CARTESIAN_POINT ( 'NONE',  ( -46.41737087459109290, -284.5138541181401024, -194.4912392918764397 ) ) ;
#12278=CARTESIAN_POINT ( 'NONE',  ( 3.962559356409089961, -272.6092366696081513, -207.8973601537884122 ) ) ;
#12279=CARTESIAN_POINT ( 'NONE',  ( -106.7679418898665773, -274.8258885968784853, -243.3615688579964456 ) ) ;
#12280=CARTESIAN_POINT ( 'NONE',  ( -93.62964140134269542, -289.3127449480446103, -221.6478562641615042 ) ) ;
#12281=CARTESIAN_POINT ( 'NONE',  ( -61.98152825431640167, -279.2293862984769248, -342.0627609226370964 ) ) ;
#12283=CARTESIAN_POINT ( 'NONE',  ( -66.06970082331426397, -279.6654330015371102, -203.2378524186758568 ) ) ;
#12284=CARTESIAN_POINT ( 'NONE',  ( 32.83476664340047080, -280.6302785096988828, -249.8878139061026786 ) ) ;
#12285=CARTESIAN_POINT ( 'NONE',  ( 36.59131022884746898, -276.8887249210343953, -290.7915417684785098 ) ) ;
#12286=CARTESIAN_POINT ( 'NONE',  ( 20.77492727107647852, -279.6698321323710843, -220.4365949994931100 ) ) ;
#12287=CARTESIAN_POINT ( 'NONE',  ( 195.1743528851788199, 283.2594845134466368, -110.5268553716196749 ) ) ;
#12288=CARTESIAN_POINT ( 'NONE',  ( -83.44836953659944356, -274.3789098938663074, -208.9187287201598622 ) ) ;
#12289=CARTESIAN_POINT ( 'NONE',  ( -43.26235011396510544, -299.4041787160501826, -194.1272658402198203 ) ) ;
#12290=CARTESIAN_POINT ( 'NONE',  ( 31.95455697924148097, -289.6233781216988064, -236.9535640164627637 ) ) ;
#12293=CARTESIAN_POINT ( 'NONE',  ( -0.8255832566043728171, -289.6350506796578088, -333.9868366128078492 ) ) ;
#12294=CARTESIAN_POINT ( 'NONE',  ( 35.71071140791632104, -289.0445011284853081, -249.2623049460595723 ) ) ;
#12295=CARTESIAN_POINT ( 'NONE',  ( -56.09973924764294395, -288.6486645537076470, -341.0680395405777858 ) ) ;
#12296=CARTESIAN_POINT ( 'NONE',  ( -111.0508255130668118, -283.7822792773383753, -292.4634374057991408 ) ) ;
#12297=CARTESIAN_POINT ( 'NONE',  ( -11.74252710806512567, -92.25804922821241405, -360.0298267093687059 ) ) ;
#12298=CARTESIAN_POINT ( 'NONE',  ( 24.36249257634518628, -279.3957484082234259, -229.7839498355443482 ) ) ;
#12299=CARTESIAN_POINT ( 'NONE',  ( -60.38415036879518283, -287.6105736046046673, -199.7926337589588286 ) ) ;
#12300=CARTESIAN_POINT ( 'NONE',  ( 26.14661009765528377, -280.5423287361759890, -307.8777115820259382 ) ) ;
#12301=CARTESIAN_POINT ( 'NONE',  ( -96.81456792384837229, -280.4675065571523191, -227.1844868604487715 ) ) ;
#12302=CARTESIAN_POINT ( 'NONE',  ( -40.50215777285083618, -277.5852773837323753, -343.3667429060195673 ) ) ;
#12303=CARTESIAN_POINT ( 'NONE',  ( -106.8934364363057625, -289.7613145279184437, -238.1323836803984477 ) ) ;
#12304=CARTESIAN_POINT ( 'NONE',  ( -108.0744848543433960, -284.9705600630828712, -300.5143860453322873 ) ) ;
#12305=CARTESIAN_POINT ( 'NONE',  ( -99.73488931745403363, -284.4460960140673933, -315.4681035871540189 ) ) ;
#12306=CARTESIAN_POINT ( 'NONE',  ( -18.73358778480818643, -282.9725910021337540, -341.0020354171684858 ) ) ;
#12309=CARTESIAN_POINT ( 'NONE',  ( -112.7793822618751278, -292.5088696306393672, -262.7844240488696528 ) ) ;
#12310=CARTESIAN_POINT ( 'NONE',  ( 12.96686980223632979, -291.4225696925302032, -212.7213221546050761 ) ) ;
#12311=CARTESIAN_POINT ( 'NONE',  ( 11.71299313959655386, -273.8116788298353868, -215.9141006872862931 ) ) ;
#12312=CARTESIAN_POINT ( 'NONE',  ( -99.93037944374245285, -295.3071608886352806, -315.1270986449532643 ) ) ;
#12313=CARTESIAN_POINT ( 'NONE',  ( -100.2939329859144948, -289.5547202451573980, -232.0502301077711138 ) ) ;
#12314=CARTESIAN_POINT ( 'NONE',  ( -41.11296538479525964, -293.3400869444051295, -344.2910536434748110 ) ) ;
#12315=CARTESIAN_POINT ( 'NONE',  ( -109.1020049645889003, -291.9594656185281565, -254.9471906481589087 ) ) ;
#12316=DIRECTION ( 'NONE',  ( 0.000000000000000000, 0.000000000000000000, -1.000000000000000000 ) ) ;
#12317=CARTESIAN_POINT ( 'NONE',  ( -51.28777609540209426, -291.2306304234671188, -344.0530959106517344 ) ) ;
#12318=CARTESIAN_POINT ( 'NONE',  ( 35.98959470203071476, -291.7642438109647287, -286.9282053159424208 ) ) ;
#12319=CARTESIAN_POINT ( 'NONE',  ( -73.85753729900216058, -297.5371780412540943, -335.8858413564130956 ) ) ;
#12320=CARTESIAN_POINT ( 'NONE',  ( -30.52126939088868696, -287.0816260456099940, -197.3931473229183950 ) ) ;
#12321=CARTESIAN_POINT ( 'NONE',  ( 27.99403419739965670, -296.0479111324673909, -307.6317697364838750 ) ) ;
#12322=CARTESIAN_POINT ( 'NONE',  ( 12.84974033404173710, -276.7279805236878474, -214.0844165269328983 ) ) ;
#12323=CARTESIAN_POINT ( 'NONE',  ( -54.54904394307327919, -297.0336317297703204, -195.4740954831521833 ) ) ;
#12324=CARTESIAN_POINT ( 'NONE',  ( -24.17099700790322103, -275.1216660739979716, -343.2453244915890309 ) ) ;
#12325=CARTESIAN_POINT ( 'NONE',  ( -57.47973599684804213, -277.8700182071046356, -198.6968053393258913 ) ) ;
#12326=CARTESIAN_POINT ( 'NONE',  ( -98.18088628750028590, -274.3258788034443683, -229.2128516132085565 ) ) ;
#12327=CARTESIAN_POINT ( 'NONE',  ( 24.85790375305440136, -273.5342227035681617, -225.9561232890435747 ) ) ;
#12328=CARTESIAN_POINT ( 'NONE',  ( -108.8674592320696632, -297.7502853114162349, -287.7185590533965751 ) ) ;
#12330=CARTESIAN_POINT ( 'NONE',  ( -109.5205565110302359, -297.1976890153803197, -282.3116166514656129 ) ) ;
#12332=CARTESIAN_POINT ( 'NONE',  ( 30.20170578519502769, -286.0123585095279850, -303.8897227860072690 ) ) ;
#12333=CARTESIAN_POINT ( 'NONE',  ( -85.30856530277549155, -273.2010595982754353, -215.2648465032376635 ) ) ;
#12334=CARTESIAN_POINT ( 'NONE',  ( -37.98244548293538259, -286.0443322566591746, -193.3637839677369072 ) ) ;
#12335=CARTESIAN_POINT ( 'NONE',  ( -105.1393533608000439, -289.7473706317709912, -306.8196218956072698 ) ) ;
#12336=CARTESIAN_POINT ( 'NONE',  ( -107.3696304866851676, -298.8943726077774841, -242.3910098301828384 ) ) ;
#12337=CARTESIAN_POINT ( 'NONE',  ( -31.48362787898167880, -292.9779849416254933, -345.0161856952290691 ) ) ;
#12338=CARTESIAN_POINT ( 'NONE',  ( 25.79180670193011693, -281.3294068004708492, -314.1828745627234412 ) ) ;
#12339=CARTESIAN_POINT ( 'NONE',  ( -4.771743288812454686, -289.9809262143061801, -202.8022627189028810 ) ) ;
#12340=CARTESIAN_POINT ( 'NONE',  ( 13.01691457970142984, -278.7548853946701115, -214.7132872792192302 ) ) ;
#12342=CARTESIAN_POINT ( 'NONE',  ( -5.634717298421447751, -287.4204732917380625, -336.5562669444793755 ) ) ;
#12343=DIRECTION ( 'NONE',  ( 0.9951408606192336803, 1.205805641958489930E-17, 0.09846150276128748380 ) ) ;
#12344=CARTESIAN_POINT ( 'NONE',  ( -102.0418455001494067, -288.0438598972423279, -308.3961917731384119 ) ) ;
#12345=CARTESIAN_POINT ( 'NONE',  ( -93.36486008588094876, -298.8288843281441132, -222.3016279232871568 ) ) ;
#12346=CARTESIAN_POINT ( 'NONE',  ( -8.246308434866241655, -284.1039444616968126, -341.0717746061306457 ) ) ;
#12347=CARTESIAN_POINT ( 'NONE',  ( -84.17406545711961030, -295.4318630093549132, -211.3260745132724026 ) ) ;
#12348=CARTESIAN_POINT ( 'NONE',  ( 28.97268187461106947, -281.1389756182431370, -239.7210847254205532 ) ) ;
#12349=CARTESIAN_POINT ( 'NONE',  ( -89.60986098759802587, -297.5063607904565970, -213.7465203535422802 ) ) ;
#12350=CARTESIAN_POINT ( 'NONE',  ( -74.58715180564381342, -274.9718270474398878, -206.8343631794590181 ) ) ;
#12351=CARTESIAN_POINT ( 'NONE',  ( -8.334658402542197919, -282.4320570626722429, -201.1836710167748379 ) ) ;
#12352=B_SPLINE_CURVE_WITH_KNOTS ( 'NONE', 3,
 ( #59600, #7981, #23117, #80413, #45817, #15097, #8447, #43957, #45342, #52465, #72855, #66687, #88901, #52000, #87053, #36875, #16034, #51525, #65790, #29782, #44430, #58661, #81339, #67162 ),
 .UNSPECIFIED., .F., .F.,
 ( 4, 2, 2, 2, 2, 2, 2, 2, 2, 2, 2, 4 ),
 ( 0.000000000000000000, 0.06250000000000000000, 0.1250000000000000000, 0.2500000000000000000, 0.3750000000000000000, 0.5000000000000000000, 0.6250000000000000000, 0.7500000000000000000, 0.8125000000000000000, 0.8750000000000000000, 0.9375000000000000000, 1.000000000000000000 ),
 .UNSPECIFIED. ) ;
#12353=CARTESIAN_POINT ( 'NONE',  ( -109.8866175390029412, -271.6157113375448944, -259.4571357085231966 ) ) ;
#12357=CARTESIAN_POINT ( 'NONE',  ( -110.5468839981672460, -286.7202603077519143, -255.7718116152337018 ) ) ;
#12359=CARTESIAN_POINT ( 'NONE',  ( 40.65961533371913106, -278.8380690714489560, -252.5904736702033802 ) ) ;
#12360=CARTESIAN_POINT ( 'NONE',  ( -100.3389879459672898, -277.1665491118436080, -314.3554420278452994 ) ) ;
#12361=CARTESIAN_POINT ( 'NONE',  ( -97.54026788375671231, -288.3216059542572793, -317.0791322641306351 ) ) ;
#12363=CARTESIAN_POINT ( 'NONE',  ( -42.96670276048308779, -284.6444194685781213, -343.8900249105404896 ) ) ;
#12364=CARTESIAN_POINT ( 'NONE',  ( 30.90695707659207514, -276.7784004215046139, -242.1456897177627070 ) ) ;
#12365=CARTESIAN_POINT ( 'NONE',  ( -113.7649760321169339, -285.9460777749832801, -272.8483026054009315 ) ) ;
#12366=CARTESIAN_POINT ( 'NONE',  ( -80.87391478423749902, -282.4525475443406890, -329.5181572540485035 ) ) ;
#12367=CARTESIAN_POINT ( 'NONE',  ( -32.86849959756012396, -282.1086894136328738, -195.4946293040974012 ) ) ;
#12368=CARTESIAN_POINT ( 'NONE',  ( -34.10531919109820365, -274.2584813910368098, -193.4291620542774695 ) ) ;
#12369=CARTESIAN_POINT ( 'NONE',  ( -111.8279815417099314, -278.1406233807484796, -289.9268728162484194 ) ) ;
#12370=CARTESIAN_POINT ( 'NONE',  ( -73.99047156523944579, -297.4632290545595197, -335.1544953516561804 ) ) ;
#12372=EDGE_CURVE ( 'NONE', #25769, #34721, #20961, .T. ) ;
#12374=CARTESIAN_POINT ( 'NONE',  ( -111.6721816342009248, -294.8790802923677461, -255.6219096070480532 ) ) ;
#12375=CARTESIAN_POINT ( 'NONE',  ( -3.844833691172875767, -276.1053555423025614, -335.2914528095027435 ) ) ;
#12376=CARTESIAN_POINT ( 'NONE',  ( -65.44160412548666272, -298.7730784402122026, -198.9468872621766025 ) ) ;
#12377=CARTESIAN_POINT ( 'NONE',  ( -44.13945563225464497, -287.7251643746256491, -196.6606123302011895 ) ) ;
#12378=CARTESIAN_POINT ( 'NONE',  ( -6.064032080916389233, -296.1686117307091308, -339.9629515513158253 ) ) ;
#12379=CARTESIAN_POINT ( 'NONE',  ( -11.17832639995599209, -295.9238376586882282, -342.4138347899152564 ) ) ;
#12380=CARTESIAN_POINT ( 'NONE',  ( -112.0781864990786971, -292.6130086766314093, -265.6448368251349734 ) ) ;
#12382=CARTESIAN_POINT ( 'NONE',  ( 14.62613770033450855, -278.7850881638697160, -216.4430617230063376 ) ) ;
#12383=CARTESIAN_POINT ( 'NONE',  ( -62.82443310092831723, -281.6381287760690952, -200.3642630252234085 ) ) ;
#12384=CARTESIAN_POINT ( 'NONE',  ( -41.13661430115381279, -293.1800999510632550, -344.7171427419654606 ) ) ;
#12385=CARTESIAN_POINT ( 'NONE',  ( -85.30188125907153562, -285.5672148244704545, -329.0137096019414571 ) ) ;
#12386=CARTESIAN_POINT ( 'NONE',  ( -91.74140396466356151, -284.1740150678466534, -221.1449300419688484 ) ) ;
#12387=CARTESIAN_POINT ( 'NONE',  ( 204.9738562182569979, 293.6303156117443223, -54.00000000000747491 ) ) ;
#12389=CARTESIAN_POINT ( 'NONE',  ( -110.2490565082685663, -284.2835098783307330, -265.4595574974268857 ) ) ;
#12391=CARTESIAN_POINT ( 'NONE',  ( 35.03138931000073342, -282.3087423848197659, -244.8327572750843615 ) ) ;
#12392=CARTESIAN_POINT ( 'NONE',  ( -78.87058298120439304, -273.8087513320262474, -210.2377325723746537 ) ) ;
#12393=CARTESIAN_POINT ( 'NONE',  ( 36.31371157666659144, -286.0797629835053044, -249.1277041300705548 ) ) ;
#12394=CARTESIAN_POINT ( 'NONE',  ( 39.04524470153614857, -282.5952721576835529, -278.4816875874217885 ) ) ;
#12395=CARTESIAN_POINT ( 'NONE',  ( -111.1518169033748933, -279.8271526880959641, -289.7715003554112627 ) ) ;
#12396=CARTESIAN_POINT ( 'NONE',  ( -67.33036735255592475, -280.3204651058207446, -199.5515661913208021 ) ) ;
#12397=CARTESIAN_POINT ( 'NONE',  ( -21.39648532958014826, -274.3380690714489560, -340.3683826091709079 ) ) ;
#12398=CARTESIAN_POINT ( 'NONE',  ( 203.3400678907170231, 292.9455748915181061, -83.20730514549673273 ) ) ;
#12400=CARTESIAN_POINT ( 'NONE',  ( -92.49043599584310016, -275.2606048649046784, -219.7590873547483170 ) ) ;
#12401=CARTESIAN_POINT ( 'NONE',  ( -112.9615723932939062, -270.7119090785686240, -296.2735061844161351 ) ) ;
#12402=CARTESIAN_POINT ( 'NONE',  ( -43.87037679853860084, -277.9894685846156790, -195.9510056702047507 ) ) ;
#12403=CARTESIAN_POINT ( 'NONE',  ( 38.21597287674843813, -295.2040146367762645, -261.8172931764508462 ) ) ;
#12404=CARTESIAN_POINT ( 'NONE',  ( -47.81583098944544474, -294.5373146293514424, -342.7601395228516026 ) ) ;
#12405=CARTESIAN_POINT ( 'NONE',  ( -109.4139899671798446, -290.4023521162516204, -243.2814220093720792 ) ) ;
#12407=CARTESIAN_POINT ( 'NONE',  ( -74.33711193959376828, -294.1084524502449540, -337.2780333952446199 ) ) ;
#12408=CARTESIAN_POINT ( 'NONE',  ( 28.37974902053175441, -285.4995115546490752, -236.6756032379166470 ) ) ;
#12409=CARTESIAN_POINT ( 'NONE',  ( 35.42259604894641001, -295.2218198698093943, -255.6566055860660640 ) ) ;
#12410=CARTESIAN_POINT ( 'NONE',  ( 29.86931596887154683, -286.6359094285825222, -300.2181546650601831 ) ) ;
#12411=CARTESIAN_POINT ( 'NONE',  ( -108.5670512060605404, -285.6298209544997917, -288.4772114669492566 ) ) ;
#12413=CARTESIAN_POINT ( 'NONE',  ( -112.4124034799732925, -291.6953305836013328, -254.2612952486399536 ) ) ;
#12414=CARTESIAN_POINT ( 'NONE',  ( 28.20905029452487156, -282.4827303476370730, -302.7418395665159210 ) ) ;
#12415=CARTESIAN_POINT ( 'NONE',  ( -113.2063622782859227, -295.4816453028025762, -259.6568538004638071 ) ) ;
#12416=CARTESIAN_POINT ( 'NONE',  ( -74.34057437189321149, -290.3340253990980955, -337.7203453135224436 ) ) ;
#12417=CARTESIAN_POINT ( 'NONE',  ( -74.39217739053599132, -290.0235901612713292, -337.8060412764365879 ) ) ;
#12418=CARTESIAN_POINT ( 'NONE',  ( 11.13247268856299321, -286.9121436349000760, -215.7106547222429072 ) ) ;
#12421=CARTESIAN_POINT ( 'NONE',  ( -113.1030561598872879, -298.4217558035367688, -269.6383386235157218 ) ) ;
#12422=CARTESIAN_POINT ( 'NONE',  ( -113.1110118654578258, -295.3715647831007232, -259.6688718474485427 ) ) ;
#12423=CARTESIAN_POINT ( 'NONE',  ( -64.89355741687893442, -278.7419500879294105, -202.5060989468545358 ) ) ;
#12425=CARTESIAN_POINT ( 'NONE',  ( -0.06976037480313371231, -274.0420208480372821, -203.0384144344906190 ) ) ;
#12426=CARTESIAN_POINT ( 'NONE',  ( -110.4951657120618052, -294.9103219988043634, -279.6744437218180792 ) ) ;
#12427=CARTESIAN_POINT ( 'NONE',  ( -70.99188594780189021, -279.3615203784351024, -336.5315832779912171 ) ) ;
#12428=CARTESIAN_POINT ( 'NONE',  ( 14.37384996976745022, -272.9283413867563581, -217.1035611763335851 ) ) ;
#12429=CIRCLE ( 'NONE', #65386, 3.491568894204821749 ) ;
#12430=CARTESIAN_POINT ( 'NONE',  ( -42.40186366650118543, -296.3224685553829545, -343.5835547771696383 ) ) ;
#12431=CARTESIAN_POINT ( 'NONE',  ( -82.14384936096338663, -298.5046164229716510, -212.2709720357035792 ) ) ;
#12433=CARTESIAN_POINT ( 'NONE',  ( -66.59824771527503628, -297.0291252575901808, -340.7349231682601953 ) ) ;
#12435=CARTESIAN_POINT ( 'NONE',  ( -34.81022065091374174, -296.0836149370950352, -195.1953032834341286 ) ) ;
#12436=CARTESIAN_POINT ( 'NONE',  ( -44.31818114722263857, -292.6131409919578346, -197.5419570256928239 ) ) ;
#12437=CARTESIAN_POINT ( 'NONE',  ( -97.04722166087842083, -288.5301040387733451, -313.3800163479940579 ) ) ;
#12439=CARTESIAN_POINT ( 'NONE',  ( 19.98582186219895718, -275.3472909304086897, -218.9692655756464035 ) ) ;
#12440=EDGE_CURVE ( 'NONE', #64930, #48357, #47411, .T. ) ;
#12441=CARTESIAN_POINT ( 'NONE',  ( -69.27061200015319287, -297.9533443617694388, -204.6904847166565844 ) ) ;
#12444=CARTESIAN_POINT ( 'NONE',  ( -79.02245826540124085, -281.4734479977473711, -207.5201611191039603 ) ) ;
#12445=CARTESIAN_POINT ( 'NONE',  ( 20.70296369716275109, -279.5597516472616348, -220.5002922571243573 ) ) ;
#12446=CARTESIAN_POINT ( 'NONE',  ( -34.30343725528067722, -276.3634805228944629, -347.1991407678876271 ) ) ;
#12447=CARTESIAN_POINT ( 'NONE',  ( -22.69972827092026435, -278.6362677321605474, -195.5273926378769431 ) ) ;
#12448=CARTESIAN_POINT ( 'NONE',  ( 32.62743136519172538, -279.1936863063045848, -242.7535163127353997 ) ) ;
#12449=CARTESIAN_POINT ( 'NONE',  ( -36.71294846266656720, -272.6349288561673347, -196.7620574869183656 ) ) ;
#12450=CARTESIAN_POINT ( 'NONE',  ( -90.13164947921488590, -279.7980435887648696, -323.7076269281154737 ) ) ;
#12453=CARTESIAN_POINT ( 'NONE',  ( -84.56886566593212251, -295.6515786158510650, -210.8332350491017166 ) ) ;
#12454=CARTESIAN_POINT ( 'NONE',  ( -5.886936586929241599, -292.4543296146415514, -200.0645569234314678 ) ) ;
#12455=CARTESIAN_POINT ( 'NONE',  ( -3.526492729702133566, -278.6070885756623738, -337.5063666857230373 ) ) ;
#12456=CARTESIAN_POINT ( 'NONE',  ( -62.68212315426065118, -271.7221775671806085, -199.7717164491168660 ) ) ;
#12458=CARTESIAN_POINT ( 'NONE',  ( -98.19926406807867636, -287.0795824094070667, -225.4902741566391171 ) ) ;
#12461=CARTESIAN_POINT ( 'NONE',  ( 27.76270265590576969, -285.0541829863706198, -233.0237446742606267 ) ) ;
#12463=CARTESIAN_POINT ( 'NONE',  ( 35.22822260306186593, -292.4955694429547748, -281.6792842409594186 ) ) ;
#12464=CARTESIAN_POINT ( 'NONE',  ( 16.89279779366137646, -284.9745043794812887, -219.6522674753275055 ) ) ;
#12466=CARTESIAN_POINT ( 'NONE',  ( 30.18445706015723218, -291.9833174569805010, -303.1184909934207781 ) ) ;
#12467=CARTESIAN_POINT ( 'NONE',  ( -104.8099393678581777, -283.4977786297754960, -234.6005336521887443 ) ) ;
#12468=CARTESIAN_POINT ( 'NONE',  ( -57.34945749769401857, -281.3897339644024100, -199.3249999978065148 ) ) ;
#12469=CARTESIAN_POINT ( 'NONE',  ( 36.30518844575019699, -288.4895252718519032, -249.0981684694154978 ) ) ;
#12470=CARTESIAN_POINT ( 'NONE',  ( 0.8838624597298744279, -278.7942357344136326, -204.6294405367410434 ) ) ;
#12471=CARTESIAN_POINT ( 'NONE',  ( 35.62999201901077129, -287.5969868136489822, -273.7598291364836314 ) ) ;
#12472=CARTESIAN_POINT ( 'NONE',  ( -99.97873118599717657, -280.5069134843076313, -231.6377465715746951 ) ) ;
#12473=CARTESIAN_POINT ( 'NONE',  ( -19.50506179501759618, -281.0901914715744851, -199.3548134191441363 ) ) ;
#12474=CARTESIAN_POINT ( 'NONE',  ( -63.98964146788656393, -287.6862320653694383, -199.8611244874135480 ) ) ;
#12475=ORIENTED_EDGE ( 'NONE', *, *, #37335, .F. ) ;
#12476=CARTESIAN_POINT ( 'NONE',  ( -34.04482923856807020, -297.9256827530350051, -193.3612081204445019 ) ) ;
#12477=CARTESIAN_POINT ( 'NONE',  ( -96.23301752009128052, -291.8998068935681545, -316.2474274031009145 ) ) ;
#12479=CARTESIAN_POINT ( 'NONE',  ( -111.2586520408596868, -292.6233781216987495, -305.9938812882205070 ) ) ;
#12481=CARTESIAN_POINT ( 'NONE',  ( 12.76187576679671487, -272.7485685143941510, -214.2588703792187346 ) ) ;
#12483=CARTESIAN_POINT ( 'NONE',  ( -47.54483155135947214, -293.5796661298963386, -345.8749347531792750 ) ) ;
#12484=CARTESIAN_POINT ( 'NONE',  ( -77.54060728728036622, -297.0045600447964489, -209.2918332226240068 ) ) ;
#12485=CARTESIAN_POINT ( 'NONE',  ( -75.05424157569694898, -291.0844731753718406, -333.6884367479887032 ) ) ;
#12486=CARTESIAN_POINT ( 'NONE',  ( 32.31580917044831835, -283.6426652404380775, -295.5288839550758553 ) ) ;
#12487=CARTESIAN_POINT ( 'NONE',  ( -95.00164907939179670, -291.2944362752274401, -320.5002901026065274 ) ) ;
#12488=CARTESIAN_POINT ( 'NONE',  ( -40.30279585126334041, -290.4037821986844392, -346.8236431289408301 ) ) ;
#12489=CARTESIAN_POINT ( 'NONE',  ( -101.3285898918744294, -287.0781584886605060, -231.1382287861074758 ) ) ;
#12490=CARTESIAN_POINT ( 'NONE',  ( -56.55870617511166643, -279.9778946840347658, -195.7426766231734234 ) ) ;
#12491=CARTESIAN_POINT ( 'NONE',  ( -112.6828941468750713, -294.7134820151158578, -263.9675006785436722 ) ) ;
#12492=CARTESIAN_POINT ( 'NONE',  ( -37.31638290146443637, -282.8851281031414260, -347.3741790559139417 ) ) ;
#12493=CARTESIAN_POINT ( 'NONE',  ( 30.28916643297933575, -277.8182393984351393, -300.9704525998034796 ) ) ;
#12494=CARTESIAN_POINT ( 'NONE',  ( -105.5795714935544112, -280.8376638359844151, -285.9686137636504668 ) ) ;
#12495=CARTESIAN_POINT ( 'NONE',  ( 26.78150406902601333, -274.3346237493449848, -311.2288291974931553 ) ) ;
#12498=CARTESIAN_POINT ( 'NONE',  ( 34.28977249104462999, -281.2502315824781363, -284.8087857765748936 ) ) ;
#12500=CARTESIAN_POINT ( 'NONE',  ( -111.4394256844100539, -279.5121573902982277, -289.8428990881785126 ) ) ;
#12501=CARTESIAN_POINT ( 'NONE',  ( -95.63002029292010775, -284.2877062388921559, -220.3285079794843853 ) ) ;
#12502=CARTESIAN_POINT ( 'NONE',  ( 17.47378833182729707, -294.6087169952544969, -220.5543350787875738 ) ) ;
#12503=CARTESIAN_POINT ( 'NONE',  ( -46.80208557936183666, -275.5340609822649185, -194.7506589084638904 ) ) ;
#12505=CARTESIAN_POINT ( 'NONE',  ( -97.43617757623091791, -274.5046614627762551, -223.0118618609506598 ) ) ;
#12507=CARTESIAN_POINT ( 'NONE',  ( 25.37448573153797682, -275.8990968957646146, -307.7199192978276869 ) ) ;
#12508=CARTESIAN_POINT ( 'NONE',  ( -97.05215672422032469, -297.9339028496198694, -315.4897544189734617 ) ) ;
#12509=CARTESIAN_POINT ( 'NONE',  ( -109.1060049771863874, -282.8278768419540370, -248.9704584469216684 ) ) ;
#12511=CARTESIAN_POINT ( 'NONE',  ( 28.03664500919741087, -292.6860013646905827, -229.6227672039093761 ) ) ;
#12512=CARTESIAN_POINT ( 'NONE',  ( 36.73520837720445087, -273.6961219794714566, -279.9623556402026452 ) ) ;
#12513=CARTESIAN_POINT ( 'NONE',  ( -12.46543918051157362, -290.3341975005167797, -342.4414945516092530 ) ) ;
#12514=CARTESIAN_POINT ( 'NONE',  ( -92.78128892305208808, -290.1530917711041297, -222.3957339172780507 ) ) ;
#12516=CARTESIAN_POINT ( 'NONE',  ( -71.88949824125222676, -290.1792740998022282, -202.1919846057980124 ) ) ;
#12517=CARTESIAN_POINT ( 'NONE',  ( -107.4143889406865355, -290.4910701331420455, -249.7763837881663846 ) ) ;
#12519=CARTESIAN_POINT ( 'NONE',  ( 37.07354313463295625, -288.3988865489286582, -251.8175454820308801 ) ) ;
#12520=CARTESIAN_POINT ( 'NONE',  ( -107.9941173629488276, -279.1295116272421524, -251.8641349634359017 ) ) ;
#12521=CARTESIAN_POINT ( 'NONE',  ( -93.47264148177617926, -294.7571209237502217, -322.6376151942385491 ) ) ;
#12522=CARTESIAN_POINT ( 'NONE',  ( -113.7193609928771423, -285.3154080728642157, -261.4299530372964000 ) ) ;
#12523=CARTESIAN_POINT ( 'NONE',  ( -111.7019020203254058, -285.1370244877222149, -250.2533294845411547 ) ) ;
#12524=CARTESIAN_POINT ( 'NONE',  ( 19.37114671263906374, -282.5362602063959798, -316.3780075690812623 ) ) ;
#12525=CARTESIAN_POINT ( 'NONE',  ( 173.9735501344063948, 243.4424551670193466, -179.7288663750133821 ) ) ;
#12526=CARTESIAN_POINT ( 'NONE',  ( -100.6629394507023250, -246.7894274234220404, -333.2501944198467072 ) ) ;
#12527=CARTESIAN_POINT ( 'NONE',  ( 44.32992207132367213, 11.63825656539217235, -328.4651697331042328 ) ) ;
#12528=CARTESIAN_POINT ( 'NONE',  ( 15.57062826419014634, -274.0214327175541484, -219.7616671598360654 ) ) ;
#12529=CARTESIAN_POINT ( 'NONE',  ( 34.46457528060756914, -274.6664670583908219, -285.1288153808118295 ) ) ;
#12530=CARTESIAN_POINT ( 'NONE',  ( -112.2473314949235146, -295.8391929396597106, -287.9872224215492906 ) ) ;
#12531=CARTESIAN_POINT ( 'NONE',  ( 26.68328070931609020, -24.59112382776695682, -341.9535762841285873 ) ) ;
#12532=CARTESIAN_POINT ( 'NONE',  ( 38.82803177079595969, -274.1398807313123598, -262.6468285325606189 ) ) ;
#12533=CARTESIAN_POINT ( 'NONE',  ( -36.75017892490402005, -275.8198262182843337, -196.3375581050478331 ) ) ;
#12535=CARTESIAN_POINT ( 'NONE',  ( -112.9699592356097213, -297.3245466989074544, -283.8212697521575478 ) ) ;
#12536=CARTESIAN_POINT ( 'NONE',  ( -5.760160217979543695, -289.1176213097603522, -336.2443083940181054 ) ) ;
#12537=AXIS2_PLACEMENT_3D ( 'NONE', #41206, #62576, #25166 ) ;
#12538=CARTESIAN_POINT ( 'NONE',  ( -114.0719024077377952, -297.2925955457415625, -275.3391217207804971 ) ) ;
#12539=CARTESIAN_POINT ( 'NONE',  ( -74.57108344939425137, -296.0257622879685755, -337.7520507797435130 ) ) ;
#12540=CARTESIAN_POINT ( 'NONE',  ( -12.26220003297685324, -292.5542633796108021, -201.7505587413596118 ) ) ;
#12542=CARTESIAN_POINT ( 'NONE',  ( 24.89496570573188805, -278.0497655484517736, -313.2992567531924237 ) ) ;
#12544=CARTESIAN_POINT ( 'NONE',  ( -3.678867409004826339, -279.9921397825090708, -201.1632268794262757 ) ) ;
#12545=ADVANCED_BREP_SHAPE_REPRESENTATION ( '', ( #58557, #18940 ), #6864 ) ;
#12546=CARTESIAN_POINT ( 'NONE',  ( -61.85733367897015000, -278.3198946977102537, -339.4251157334522873 ) ) ;
#12547=CARTESIAN_POINT ( 'NONE',  ( 38.30620234176479499, -277.2147004842683486, -262.6604537507460577 ) ) ;
#12548=CARTESIAN_POINT ( 'NONE',  ( -99.13156550678466772, -275.9896795546921453, -313.4936966241423306 ) ) ;
#12549=CARTESIAN_POINT ( 'NONE',  ( -110.3430300130309263, -297.1530649146155270, -274.1949806450746223 ) ) ;
#12550=CARTESIAN_POINT ( 'NONE',  ( -78.29258560499850716, -294.1893375310316969, -331.5651323288159347 ) ) ;
#12552=CARTESIAN_POINT ( 'NONE',  ( -33.92428390281050099, -280.5864098914588567, -193.4985902482769973 ) ) ;
#12554=CARTESIAN_POINT ( 'NONE',  ( 9.665668289305965999, -276.5505233591932779, -326.2118773234645346 ) ) ;
#12555=CARTESIAN_POINT ( 'NONE',  ( 29.70750037557199263, -285.7554731685211209, -233.4041290271505034 ) ) ;
#12556=CARTESIAN_POINT ( 'NONE',  ( -34.16995150064371245, -300.0919240008499855, -195.1933642773144300 ) ) ;
#12557=CARTESIAN_POINT ( 'NONE',  ( 82.64619460822838448, -299.7668101228608748, -197.8578870376357202 ) ) ;
#12559=CARTESIAN_POINT ( 'NONE',  ( 19.63281298001173880, -287.3968030300295027, -316.2578126745939358 ) ) ;
#12560=CARTESIAN_POINT ( 'NONE',  ( -49.28363519112350843, -278.1377146732341430, -197.3175405894177459 ) ) ;
#12561=CARTESIAN_POINT ( 'NONE',  ( -46.51203322022012543, -278.5083584211845391, -197.2939903880773329 ) ) ;
#12562=CARTESIAN_POINT ( 'NONE',  ( -34.82181443857170677, -281.1001297837638049, -344.7711413711398905 ) ) ;
#12563=CARTESIAN_POINT ( 'NONE',  ( -42.90293920771659231, -287.9821445867680723, -195.5548116255564253 ) ) ;
#12564=CARTESIAN_POINT ( 'NONE',  ( -93.90226149250428023, -279.0974685749752666, -317.1572238003803363 ) ) ;
#12567=CARTESIAN_POINT ( 'NONE',  ( -83.06769276739125019, -293.4268758816918421, -210.8470617778256440 ) ) ;
#12569=CARTESIAN_POINT ( 'NONE',  ( -35.75543595774144023, -275.2724075324279625, -346.3441802229037307 ) ) ;
#12570=TOROIDAL_SURFACE ( 'NONE', #76095, 5.654241149514406040, 1.000000000000000000 ) ;
#12571=CARTESIAN_POINT ( 'NONE',  ( 28.12548131681101893, -276.6453486622205560, -303.0012608549447464 ) ) ;
#12572=CARTESIAN_POINT ( 'NONE',  ( 33.88036123089335661, -283.8642270593254011, -294.5531513830283075 ) ) ;
#12574=DIRECTION ( 'NONE',  ( -1.000000000000000000, -0.000000000000000000, -0.000000000000000000 ) ) ;
#12575=CARTESIAN_POINT ( 'NONE',  ( -71.23814853932458391, -291.4163005853861819, -337.8914444056980528 ) ) ;
#12577=CARTESIAN_POINT ( 'NONE',  ( -108.1215329218913581, -294.8749532840054712, -245.4043380101404352 ) ) ;
#12578=CARTESIAN_POINT ( 'NONE',  ( -54.91772352308628058, -285.0288881253230784, -195.5597662460230310 ) ) ;
#12580=CARTESIAN_POINT ( 'NONE',  ( 24.21564609138414426, -273.6843904535077172, -230.2121876813570793 ) ) ;
#12581=CARTESIAN_POINT ( 'NONE',  ( 35.27090687749453224, -291.8927658334631019, -285.8581534860165903 ) ) ;
#12582=FACE_OUTER_BOUND ( 'NONE', #53992, .T. ) ;
#12584=CARTESIAN_POINT ( 'NONE',  ( -96.03307207509081422, -289.6939516939546593, -221.5758770953208909 ) ) ;
#12585=CARTESIAN_POINT ( 'NONE',  ( -105.9502146030623777, -285.7908552118423131, -297.6904242434161461 ) ) ;
#12586=CARTESIAN_POINT ( 'NONE',  ( 38.62744524904720578, -285.7713300987560956, -268.7292595337831358 ) ) ;
#12588=CARTESIAN_POINT ( 'NONE',  ( -91.97073117390672792, -286.6785543492987927, -220.9806032714806463 ) ) ;
#12589=CARTESIAN_POINT ( 'NONE',  ( -2.117599204566144255, -287.3336202621802613, -206.1804585664824003 ) ) ;
#12590=CARTESIAN_POINT ( 'NONE',  ( -70.20369978855059401, -293.6011619459533222, -202.5489082699899370 ) ) ;
#12591=CARTESIAN_POINT ( 'NONE',  ( 35.49094456198201897, -273.8893841493771788, -290.5269593316224359 ) ) ;
#12592=CARTESIAN_POINT ( 'NONE',  ( 33.69239798872150260, -275.5065372135939583, -240.5603346329096155 ) ) ;
#12593=CARTESIAN_POINT ( 'NONE',  ( -40.54640512744872893, -290.0920261457404195, -194.8561688827246599 ) ) ;
#12594=CARTESIAN_POINT ( 'NONE',  ( -79.91078213175143219, -279.4938746968505825, -206.1342929073309449 ) ) ;
#12595=CARTESIAN_POINT ( 'NONE',  ( -111.8556681748940349, -298.5890412720779068, -265.9434980272143889 ) ) ;
#12598=CARTESIAN_POINT ( 'NONE',  ( -110.4834773936178607, -283.3375926751205043, -262.6819869511061825 ) ) ;
#12599=CARTESIAN_POINT ( 'NONE',  ( -70.33130833008823402, -277.6171799092439301, -203.0061894027116693 ) ) ;
#12601=CARTESIAN_POINT ( 'NONE',  ( -27.07050527769958137, -272.6602060880990734, -194.6959316172027457 ) ) ;
#12602=CARTESIAN_POINT ( 'NONE',  ( -53.98518798882874847, -276.6199614661547344, -341.5954021164458254 ) ) ;
#12603=CARTESIAN_POINT ( 'NONE',  ( 33.42131565614240429, -295.3424034750860301, -290.9808527754635179 ) ) ;
#12604=CONICAL_SURFACE ( 'NONE', #27751, 2.738891987356051327, 0.09862129276975473147 ) ;
#12605=CARTESIAN_POINT ( 'NONE',  ( -36.74111090155958692, -278.9798690578548985, -193.6595869428859373 ) ) ;
#12606=CARTESIAN_POINT ( 'NONE',  ( -86.63954514880765601, -296.6990598476846799, -324.5195053651119679 ) ) ;
#12607=CARTESIAN_POINT ( 'NONE',  ( -97.01221858130472242, -297.2213807722670253, -318.2642803681642931 ) ) ;
#12608=CARTESIAN_POINT ( 'NONE',  ( -66.81739334731882707, -297.4881823881186165, -203.5628329864630928 ) ) ;
#12609=CARTESIAN_POINT ( 'NONE',  ( -19.62372796187571566, -294.2800220444470938, -197.4303042952196563 ) ) ;
#12610=CARTESIAN_POINT ( 'NONE',  ( -111.7217710860096389, -284.9704502704320248, -250.2457526416982319 ) ) ;
#12611=CARTESIAN_POINT ( 'NONE',  ( 26.59355548651324597, -274.2343652001097780, -311.1106352812315663 ) ) ;
#12612=CARTESIAN_POINT ( 'NONE',  ( 27.44364859138365986, -287.9325248714616237, -312.0750310898934003 ) ) ;
#12613=CARTESIAN_POINT ( 'NONE',  ( -88.67975864015495802, -281.3078126908787340, -216.1024819155032901 ) ) ;
#12614=CARTESIAN_POINT ( 'NONE',  ( -72.47639672715835957, -284.6337607506645782, -206.0898606211825381 ) ) ;
#12615=CARTESIAN_POINT ( 'NONE',  ( -91.35361185486713964, -289.2840923545999203, -218.2515613434582065 ) ) ;
#12616=CARTESIAN_POINT ( 'NONE',  ( 189.0118003482855613, 275.4351431090623237, -122.7278359107281887 ) ) ;
#12617=CARTESIAN_POINT ( 'NONE',  ( 35.51273965628178075, -287.1406200928090016, -276.4927356085705128 ) ) ;
#12619=CARTESIAN_POINT ( 'NONE',  ( 37.32232758360850511, -282.7177957728447382, -288.2526722765618388 ) ) ;
#12620=CARTESIAN_POINT ( 'NONE',  ( -79.45528720899983455, -290.5574938977147212, -206.1160746953016769 ) ) ;
#12621=CARTESIAN_POINT ( 'NONE',  ( -59.09347548110813619, -281.3753634609538494, -197.3316671921994896 ) ) ;
#12622=CARTESIAN_POINT ( 'NONE',  ( -67.18563426773714298, -280.9841186722829320, -199.9151254167732930 ) ) ;
#12623=CARTESIAN_POINT ( 'NONE',  ( 20.51722863426464016, -280.7587912809323711, -225.8285062069620039 ) ) ;
#12624=CARTESIAN_POINT ( 'NONE',  ( 37.60176673436281192, -277.6041177088840186, -274.3954965778123096 ) ) ;
#12625=CARTESIAN_POINT ( 'NONE',  ( -96.51141804342559283, -295.8891836041329952, -319.6557963897648733 ) ) ;
#12626=CARTESIAN_POINT ( 'NONE',  ( -111.6068495014022801, -288.6692574196476926, -262.8421825658129478 ) ) ;
#12628=CARTESIAN_POINT ( 'NONE',  ( -75.35923858213155313, -296.4530220869546611, -207.6213878589962860 ) ) ;
#12631=CARTESIAN_POINT ( 'NONE',  ( -67.11346878464723886, -285.3656372158049521, -338.6021921623116100 ) ) ;
#12632=CARTESIAN_POINT ( 'NONE',  ( -104.7801134663028648, -296.5942811263462886, -242.3584771585584292 ) ) ;
#12634=CARTESIAN_POINT ( 'NONE',  ( 13.06492628264923717, -293.8170295869656456, -212.5626359711301347 ) ) ;
#12635=CARTESIAN_POINT ( 'NONE',  ( -58.97038684478827264, -283.9907842108303271, -340.2433558536980058 ) ) ;
#12636=CARTESIAN_POINT ( 'NONE',  ( 2.306766587584209383, -273.6284961275996466, -204.6281787519848194 ) ) ;
#12637=CARTESIAN_POINT ( 'NONE',  ( -107.1713513255442649, -291.6175047298950176, -238.0296777572972644 ) ) ;
#12638=CARTESIAN_POINT ( 'NONE',  ( -36.55408705261230295, -284.2015279658127724, -194.5875779140718578 ) ) ;
#12639=CARTESIAN_POINT ( 'NONE',  ( -109.8442033155404971, -290.5570573798880787, -296.3866958251232973 ) ) ;
#12641=CARTESIAN_POINT ( 'NONE',  ( 34.98190542943792991, -288.0194236988548369, -280.5211343545892078 ) ) ;
#12642=LINE ( 'NONE', #14519, #26290 ) ;
#12643=AXIS2_PLACEMENT_3D ( 'NONE', #42105, #72872, #7996 ) ;
#12645=CARTESIAN_POINT ( 'NONE',  ( 198.7186473392949324, 285.8615890216420894, -96.28303562970221208 ) ) ;
#12646=CARTESIAN_POINT ( 'NONE',  ( -38.70061381994710104, -284.5890215064887343, -346.6556859975646603 ) ) ;
#12647=CARTESIAN_POINT ( 'NONE',  ( 21.27581636871891391, -291.6952119285919025, -317.1477375740089997 ) ) ;
#12649=CARTESIAN_POINT ( 'NONE',  ( 12.11514108265188483, -281.2648853495474555, -324.4743966704918989 ) ) ;
#12650=CARTESIAN_POINT ( 'NONE',  ( 26.04705649364418818, -275.7966940058047953, -314.1295641626779229 ) ) ;
#12651=CARTESIAN_POINT ( 'NONE',  ( -102.1583477803547169, -280.0508082361629363, -307.8660742968231716 ) ) ;
#12652=CARTESIAN_POINT ( 'NONE',  ( -75.49606648588520841, -209.3771256275476276, -355.3995788168579111 ) ) ;
#12653=CARTESIAN_POINT ( 'NONE',  ( 34.77762986152587388, -279.8042023697440186, -244.9560258808108415 ) ) ;
#12654=CARTESIAN_POINT ( 'NONE',  ( -109.9599198805907889, -282.7957885906049000, -253.0307059700666628 ) ) ;
#12656=CARTESIAN_POINT ( 'NONE',  ( -108.4808413058894132, -297.9682693022463695, -297.2151912524603290 ) ) ;
#12658=CARTESIAN_POINT ( 'NONE',  ( 14.91514181625562330, -293.3056538800829003, -219.2278077630834048 ) ) ;
#12660=CARTESIAN_POINT ( 'NONE',  ( -52.45493329255374704, -290.5394774719989073, -198.3864549677211073 ) ) ;
#12661=CARTESIAN_POINT ( 'NONE',  ( 1.003413464882473294, -277.2061890039088325, -337.0770896462618111 ) ) ;
#12662=CARTESIAN_POINT ( 'NONE',  ( -60.51791045767454591, -297.9098365572439775, -201.0843626165640501 ) ) ;
#12665=CARTESIAN_POINT ( 'NONE',  ( -81.06283476543683264, -272.3941941989601219, -207.2891952767791111 ) ) ;
#12666=DIRECTION ( 'NONE',  ( 0.000000000000000000, 0.000000000000000000, -1.000000000000000000 ) ) ;
#12669=EDGE_CURVE ( 'NONE', #31408, #10505, #9570, .T. ) ;
#12672=CARTESIAN_POINT ( 'NONE',  ( 33.62620332539215440, -282.8740246278042036, -288.7900241679112696 ) ) ;
#12673=CARTESIAN_POINT ( 'NONE',  ( 38.62658439766818930, -283.2706922622728030, -267.0784978993007712 ) ) ;
#12674=CARTESIAN_POINT ( 'NONE',  ( -76.26229071936403159, -282.6447775006108714, -332.4581522303788006 ) ) ;
#12675=CARTESIAN_POINT ( 'NONE',  ( 33.91367453616346950, -283.1417020225867418, -249.5395651381631126 ) ) ;
#12676=CARTESIAN_POINT ( 'NONE',  ( -1.146417747012285604, -275.0428483524368630, -334.6108277334010381 ) ) ;
#12678=CARTESIAN_POINT ( 'NONE',  ( -100.9929541079603297, -274.1292678856114549, -233.8894580073142606 ) ) ;
#12680=CARTESIAN_POINT ( 'NONE',  ( -103.4616172954073505, -278.8427701030904018, -309.6102358343944729 ) ) ;
#12684=CARTESIAN_POINT ( 'NONE',  ( -31.01105954805349896, -287.9917252804136183, -194.8481791191904904 ) ) ;
#12685=CARTESIAN_POINT ( 'NONE',  ( 6.781745895150870673, -291.8673093068106823, -212.0025433129018211 ) ) ;
#12687=CARTESIAN_POINT ( 'NONE',  ( 16.60852260737198804, -287.6580931582129210, -325.2319275647414543 ) ) ;
#12688=CARTESIAN_POINT ( 'NONE',  ( -46.83290882217585249, -284.1699898011024175, -196.9073841552745137 ) ) ;
#12689=CARTESIAN_POINT ( 'NONE',  ( -103.5506706064534086, -282.6941346864935554, -302.5990274579521611 ) ) ;
#12690=CARTESIAN_POINT ( 'NONE',  ( 10.75701678634182734, -286.6167590674494932, -326.6826433891713464 ) ) ;
#12691=CARTESIAN_POINT ( 'NONE',  ( -97.85104321354928913, -285.1810060938734637, -311.9918183803483771 ) ) ;
#12692=CARTESIAN_POINT ( 'NONE',  ( 22.74954937165943392, -274.1649601502861060, -315.2392015557825857 ) ) ;
#12693=CARTESIAN_POINT ( 'NONE',  ( -26.71232985919517944, -284.5849339588338012, -194.8531745398550186 ) ) ;
#12694=CARTESIAN_POINT ( 'NONE',  ( -105.9539577227053826, -298.9505159662763276, -239.9446853690348576 ) ) ;
#12695=CARTESIAN_POINT ( 'NONE',  ( -10.62127270455772710, -284.3995729523576870, -200.0486533792515615 ) ) ;
#12697=CARTESIAN_POINT ( 'NONE',  ( 35.93841738125772878, -282.5058196220105060, -271.3048669382784510 ) ) ;
#12698=CARTESIAN_POINT ( 'NONE',  ( 37.52611708050940109, -289.4593949972093014, -263.1082099610706564 ) ) ;
#12701=CARTESIAN_POINT ( 'NONE',  ( -3.844741996609786661, -296.5339779675770160, -338.1048239028524449 ) ) ;
#12702=CARTESIAN_POINT ( 'NONE',  ( 3.822411524978964970, -278.6056800016013995, -207.6049561217071755 ) ) ;
#12703=CARTESIAN_POINT ( 'NONE',  ( -113.5046801578881599, -289.8816134664136257, -259.8053904173704609 ) ) ;
#12704=CARTESIAN_POINT ( 'NONE',  ( -73.71424022065239967, -293.9435149377666789, -334.5754368140970314 ) ) ;
#12705=CARTESIAN_POINT ( 'NONE',  ( -99.87861719279139550, -277.7669087314573062, -231.6586605190708781 ) ) ;
#12706=CARTESIAN_POINT ( 'NONE',  ( -37.12257269282081751, -296.1945163819850109, -196.1230835325061435 ) ) ;
#12707=CARTESIAN_POINT ( 'NONE',  ( 35.91734243256483694, -294.9441356797200910, -276.2225307994201557 ) ) ;
#12708=CARTESIAN_POINT ( 'NONE',  ( -106.6379572354042153, -298.6233781216988064, -303.7686719486574134 ) ) ;
#12709=CARTESIAN_POINT ( 'NONE',  ( -57.19053941056941426, -296.2805962430873592, -196.6264160508500822 ) ) ;
#12710=CARTESIAN_POINT ( 'NONE',  ( -33.56698644350797167, -290.3389179041185457, -194.4682622474768721 ) ) ;
#12711=CARTESIAN_POINT ( 'NONE',  ( -110.2866629565564267, -292.1095333635684028, -260.2661270485664318 ) ) ;
#12713=CARTESIAN_POINT ( 'NONE',  ( -25.39276830906507243, -293.0110508689361950, -198.1304107910130767 ) ) ;
#12715=CARTESIAN_POINT ( 'NONE',  ( -84.03651937796948346, -292.6319190584698617, -209.5686206708755321 ) ) ;
#12716=CARTESIAN_POINT ( 'NONE',  ( 33.78377332379238851, -279.2496718533679996, -245.3138771476903912 ) ) ;
#12717=CARTESIAN_POINT ( 'NONE',  ( -9.727477383730715133, -292.4230616058530359, -202.7317849118470576 ) ) ;
#12719=CARTESIAN_POINT ( 'NONE',  ( 29.28658259053174007, -281.0502294714270306, -231.7648494845747962 ) ) ;
#12720=CARTESIAN_POINT ( 'NONE',  ( -34.48400638747325075, -282.6838719749498523, -347.2869126035777185 ) ) ;
#12721=CARTESIAN_POINT ( 'NONE',  ( -73.26066703526196022, -287.5294987995197289, -336.0106133696477855 ) ) ;
#12722=CARTESIAN_POINT ( 'NONE',  ( -10.55175458754369444, -280.8386386964761527, -339.6482790735918798 ) ) ;
#12723=CARTESIAN_POINT ( 'NONE',  ( -33.92675524242982732, -278.5742659129874141, -194.1309014981059988 ) ) ;
#12725=CARTESIAN_POINT ( 'NONE',  ( -36.55473865310689519, -284.9821459890060282, -193.6612795405494580 ) ) ;
#12727=CARTESIAN_POINT ( 'NONE',  ( 35.69659821302300884, -295.0142856207962154, -259.7853253038214234 ) ) ;
#12728=CARTESIAN_POINT ( 'NONE',  ( 9.137444172736250536, -276.1016893901243066, -209.7121655071458122 ) ) ;
#12729=CARTESIAN_POINT ( 'NONE',  ( -110.4131071039217176, -278.2152713700334061, -270.6338982105727382 ) ) ;
#12730=CARTESIAN_POINT ( 'NONE',  ( -108.7976714184257361, -290.3547422290420741, -299.0498644076387791 ) ) ;
#12732=CARTESIAN_POINT ( 'NONE',  ( -101.7045171753228772, -282.1048300662653787, -309.9432096195405961 ) ) ;
#12733=CARTESIAN_POINT ( 'NONE',  ( 0.03942425826137266331, -291.6217399924299798, -207.3844557355665188 ) ) ;
#12734=CARTESIAN_POINT ( 'NONE',  ( -95.86329552514342822, -293.9065832499758244, -317.2879913062499213 ) ) ;
#12738=CARTESIAN_POINT ( 'NONE',  ( -77.28356070118236687, -291.0080949154977361, -209.1840290069833088 ) ) ;
#12740=CARTESIAN_POINT ( 'NONE',  ( -6.941161984400256557, -277.9809262143061233, -207.3071070584150277 ) ) ;
#12741=CARTESIAN_POINT ( 'NONE',  ( -110.9930382571182292, -295.3381014873089612, -292.0477620371522107 ) ) ;
#12742=CARTESIAN_POINT ( 'NONE',  ( -6.707720012253735042, -278.5896021565122282, -201.0515836639664826 ) ) ;
#12743=CARTESIAN_POINT ( 'NONE',  ( -85.77714865942333233, -285.0220606485902977, -329.5836271914230338 ) ) ;
#12744=CARTESIAN_POINT ( 'NONE',  ( 9.032126467930954306, -286.5429111326134830, -213.9832126354646391 ) ) ;
#12745=CARTESIAN_POINT ( 'NONE',  ( 5.818377028963960917, -277.9756536651902366, -330.1561749321234061 ) ) ;
#12746=CARTESIAN_POINT ( 'NONE',  ( -110.8923452054956300, -294.7365372722920256, -257.6273277775270572 ) ) ;
#12747=CARTESIAN_POINT ( 'NONE',  ( -56.03793337859627144, -297.0562554884706401, -342.0272453920001112 ) ) ;
#12749=CARTESIAN_POINT ( 'NONE',  ( -61.93726522194137374, -276.1739129192278597, -339.5685261531830292 ) ) ;
#12752=CARTESIAN_POINT ( 'NONE',  ( -105.9407881765222470, -295.7676562329083367, -305.4057536379166891 ) ) ;
#12753=CARTESIAN_POINT ( 'NONE',  ( -99.29584816917089540, -291.9102256989351076, -311.6517058737210846 ) ) ;
#12756=CARTESIAN_POINT ( 'NONE',  ( -68.79432972687121151, -290.1283612228955349, -336.3506986745339304 ) ) ;
#12758=CARTESIAN_POINT ( 'NONE',  ( -48.07399228421011372, -278.9776893724890101, -194.2966627046170345 ) ) ;
#12759=CARTESIAN_POINT ( 'NONE',  ( -112.2046537130600967, -296.9827680700414589, -287.9922031837843974 ) ) ;
#12760=CARTESIAN_POINT ( 'NONE',  ( -71.59233948002955117, -289.7442008569637437, -202.7656983099762442 ) ) ;
#12761=CARTESIAN_POINT ( 'NONE',  ( -26.21778484358500450, -298.5211383845050932, -193.3816517618556645 ) ) ;
#12762=CARTESIAN_POINT ( 'NONE',  ( 12.91463599043121313, -293.1108799237808284, -217.3857636499863588 ) ) ;
#12765=CARTESIAN_POINT ( 'NONE',  ( -7.176037701193298979, -290.1837073577079877, -340.4661767328307747 ) ) ;
#12766=CARTESIAN_POINT ( 'NONE',  ( -99.86837403722181250, -280.4090924074130839, -320.2651865833026363 ) ) ;
#12768=CARTESIAN_POINT ( 'NONE',  ( 10.76571107480143397, -280.0456659282253327, -210.3012804972890990 ) ) ;
#12769=CARTESIAN_POINT ( 'NONE',  ( -98.87766549156962981, -287.1312837310651389, -227.7549693876415802 ) ) ;
#12770=CARTESIAN_POINT ( 'NONE',  ( 17.93786329305483918, -285.3993143061658770, -217.5327653407140929 ) ) ;
#12771=CARTESIAN_POINT ( 'NONE',  ( -88.57024709705110865, -271.3319616237362766, -215.7405433434926749 ) ) ;
#12772=CARTESIAN_POINT ( 'NONE',  ( -27.11609820263379333, -276.1031604155282366, -196.5748878261711923 ) ) ;
#12773=CARTESIAN_POINT ( 'NONE',  ( -110.3558600276854662, -288.4435754079615890, -284.9263076712960583 ) ) ;
#12774=CARTESIAN_POINT ( 'NONE',  ( 38.15176543325043923, -277.4939952727524428, -276.7675316607811169 ) ) ;
#12776=CARTESIAN_POINT ( 'NONE',  ( -108.1720813378868229, -278.3184213534494802, -288.0777871115324160 ) ) ;
#12777=CARTESIAN_POINT ( 'NONE',  ( -19.50166052244104620, -279.6361796699416686, -199.4171059962247057 ) ) ;
#12778=CARTESIAN_POINT ( 'NONE',  ( -45.60259956673103687, -278.2340497529474987, -346.6586354221760757 ) ) ;
#12779=CARTESIAN_POINT ( 'NONE',  ( -99.91572761369815225, -277.9348204407071421, -226.1740180188839986 ) ) ;
#12780=CARTESIAN_POINT ( 'NONE',  ( -107.8763801708993384, -260.0240351709692845, -316.1980822346592390 ) ) ;
#12781=CARTESIAN_POINT ( 'NONE',  ( -10.44133255412179473, -275.3358280256182411, -198.4074893679850788 ) ) ;
#12783=CARTESIAN_POINT ( 'NONE',  ( -31.97937589946915793, -299.5433120510044205, -193.9490722229001847 ) ) ;
#12785=CARTESIAN_POINT ( 'NONE',  ( -85.28047601435908120, -292.1948066931273615, -330.5268031993605859 ) ) ;
#12789=CARTESIAN_POINT ( 'NONE',  ( 12.37549240880803225, -289.4201731558272286, -324.3042861944137485 ) ) ;
#12790=CARTESIAN_POINT ( 'NONE',  ( 26.27695026892089913, -288.7590823455798841, -228.8082440162733349 ) ) ;
#12791=CARTESIAN_POINT ( 'NONE',  ( -23.77438266417697221, -288.2229187652478117, -342.2447789095239727 ) ) ;
#12792=CARTESIAN_POINT ( 'NONE',  ( -102.4630494542463595, -284.5967666444706197, -229.3887277045673159 ) ) ;
#12793=CARTESIAN_POINT ( 'NONE',  ( 18.58395493326880654, -279.2735022965443932, -222.1881921483092697 ) ) ;
#12794=CARTESIAN_POINT ( 'NONE',  ( -42.78799873117153396, -287.8431525050246478, -196.3131295468711812 ) ) ;
#12795=CARTESIAN_POINT ( 'NONE',  ( 34.13273993873682599, -279.7967935555730037, -252.3623101591499562 ) ) ;
#12796=CARTESIAN_POINT ( 'NONE',  ( -108.7729123399310396, -280.0938733723111227, -253.0745509007568046 ) ) ;
#12797=CARTESIAN_POINT ( 'NONE',  ( -76.38340974404744088, -278.0816915890506493, -332.1760475079382786 ) ) ;
#12798=CARTESIAN_POINT ( 'NONE',  ( 14.32451743060643601, -287.1402686412513958, -326.9892462897971654 ) ) ;
#12799=CARTESIAN_POINT ( 'NONE',  ( -0.4439788245232155206, -283.3773613274281615, -337.7757075228396388 ) ) ;
#12800=CARTESIAN_POINT ( 'NONE',  ( -52.89903591155184870, -283.7386127523722053, -345.7647274539809814 ) ) ;
#12801=CARTESIAN_POINT ( 'NONE',  ( 34.56672463139790352, -281.5529226777233589, -257.7842164114974253 ) ) ;
#12805=CARTESIAN_POINT ( 'NONE',  ( -95.64379628515675336, -293.0739427394873360, -221.9554113389173722 ) ) ;
#12806=CARTESIAN_POINT ( 'NONE',  ( 8.568464601607562514, -291.3508187861314696, -209.0940478909424485 ) ) ;
#12808=CARTESIAN_POINT ( 'NONE',  ( 35.83640159367509170, -274.6631786878368757, -274.3373165245678251 ) ) ;
#12810=CARTESIAN_POINT ( 'NONE',  ( -13.82111854622414171, -294.1033084075639863, -343.5737878452090968 ) ) ;
#12811=CARTESIAN_POINT ( 'NONE',  ( -85.14939795273411960, -288.2058409473071379, -326.5099619300196423 ) ) ;
#12812=CARTESIAN_POINT ( 'NONE',  ( 23.43264825056165179, -291.2110688170663479, -228.0959965685837290 ) ) ;
#12813=CARTESIAN_POINT ( 'NONE',  ( -95.25444729854719128, -291.1251159771306902, -315.4729269737616733 ) ) ;
#12815=CARTESIAN_POINT ( 'NONE',  ( -111.6871824480867019, -292.6841544288588466, -260.0930899425639495 ) ) ;
#12816=CARTESIAN_POINT ( 'NONE',  ( -112.1789260973729512, -288.6489151968917781, -262.7955414915831511 ) ) ;
#12817=CARTESIAN_POINT ( 'NONE',  ( 18.97023693299322389, -294.8637363602957748, -220.8045126366333477 ) ) ;
#12818=CARTESIAN_POINT ( 'NONE',  ( 0.2792775019406475434, -287.5074061434601731, -207.4683283593129488 ) ) ;
#12819=CARTESIAN_POINT ( 'NONE',  ( 14.23956241590369665, -296.3295367544030796, -325.0365400558924875 ) ) ;
#12821=CARTESIAN_POINT ( 'NONE',  ( 1.547107284693248319, -276.5491691831819594, -205.8160371446255397 ) ) ;
#12823=CARTESIAN_POINT ( 'NONE',  ( -40.42352086366273767, -297.2116406593179931, -193.5324033616849420 ) ) ;
#12824=CARTESIAN_POINT ( 'NONE',  ( -16.11134798781873556, -275.0138508440573446, -341.3179334723345164 ) ) ;
#12825=CARTESIAN_POINT ( 'NONE',  ( -41.09990449428941872, -278.0843240821507152, -196.0160435026627681 ) ) ;
#12826=CARTESIAN_POINT ( 'NONE',  ( -96.61105071479227036, -274.3611641720453349, -226.9837623274275984 ) ) ;
#12829=CARTESIAN_POINT ( 'NONE',  ( -92.62139973357824374, -297.2895323889403585, -318.9361087662082923 ) ) ;
#12830=CARTESIAN_POINT ( 'NONE',  ( -98.86356132045459333, -296.8071256839359080, -310.0476217724072967 ) ) ;
#12832=CARTESIAN_POINT ( 'NONE',  ( 37.45469921927907109, -285.6946673156867291, -279.9396689795746056 ) ) ;
#12833=CARTESIAN_POINT ( 'NONE',  ( -57.90478048487656793, -297.7790149154793653, -200.3171337566467400 ) ) ;
#12834=CARTESIAN_POINT ( 'NONE',  ( 18.35149761149446945, -286.8243567422333626, -217.1121641910426092 ) ) ;
#12835=CARTESIAN_POINT ( 'NONE',  ( -41.76358626444396549, -288.7731194933020902, -347.2260848123033270 ) ) ;
#12836=CARTESIAN_POINT ( 'NONE',  ( -67.54193801458228563, -299.6379745472079321, -201.2667484842886836 ) ) ;
#12837=CARTESIAN_POINT ( 'NONE',  ( -45.31066793678635918, -293.1530363351437813, -344.8206848949831738 ) ) ;
#12838=CARTESIAN_POINT ( 'NONE',  ( 24.46794854450271117, -280.1414208134771116, -224.7132686151190342 ) ) ;
#12839=CARTESIAN_POINT ( 'NONE',  ( -4.771743288812454686, -283.9809262143061233, -202.8022627189028810 ) ) ;
#12841=CARTESIAN_POINT ( 'NONE',  ( 22.27530300331472546, -286.9423534689038888, -313.1740067325638961 ) ) ;
#12843=CARTESIAN_POINT ( 'NONE',  ( -56.60315071815340104, -287.3001343420163494, -342.8995813082674431 ) ) ;
#12844=CARTESIAN_POINT ( 'NONE',  ( -41.93830527140335107, -299.5933930275830903, -196.7044031693784234 ) ) ;
#12845=CARTESIAN_POINT ( 'NONE',  ( 3.491637004783563647, -282.0146376710927711, -205.7134519838564870 ) ) ;
#12846=CARTESIAN_POINT ( 'NONE',  ( -54.20210191688631340, -295.8567615428426052, -196.9163519930568498 ) ) ;
#12847=CARTESIAN_POINT ( 'NONE',  ( 17.60485798695175319, -282.2378917936061953, -318.4222847527424847 ) ) ;
#12848=CARTESIAN_POINT ( 'NONE',  ( -84.18352103965089839, -295.8426409876597063, -331.5417106358412411 ) ) ;
#12849=CARTESIAN_POINT ( 'NONE',  ( -110.7781188841123310, -274.0490587354074137, -264.8875579083942284 ) ) ;
#12850=CARTESIAN_POINT ( 'NONE',  ( 37.36559402475907632, -285.4866337887550571, -258.9551431836123925 ) ) ;
#12851=CARTESIAN_POINT ( 'NONE',  ( 28.94201066895371000, -283.0857735435578206, -235.1581556957312102 ) ) ;
#12852=CARTESIAN_POINT ( 'NONE',  ( -37.13695615579317888, -297.1135314523854163, -197.1229975639101610 ) ) ;
#12855=CARTESIAN_POINT ( 'NONE',  ( -108.5474871138090549, -286.2417338954609818, -292.7571601043123337 ) ) ;
#12857=CARTESIAN_POINT ( 'NONE',  ( -2.659677404128736544, -274.1237833571632905, -342.4524372437778652 ) ) ;
#12858=CARTESIAN_POINT ( 'NONE',  ( 39.15757917469888127, -274.6521396190461246, -262.6068260781826780 ) ) ;
#12859=CARTESIAN_POINT ( 'NONE',  ( -67.79925558043403555, -291.4742574353348914, -204.0048084319964516 ) ) ;
#12860=CARTESIAN_POINT ( 'NONE',  ( -65.56348126283084810, -284.9481178865611355, -338.4500877506414440 ) ) ;
#12861=CARTESIAN_POINT ( 'NONE',  ( 34.95230614102256794, -277.3458333096415913, -285.1940905349864011 ) ) ;
#12862=CARTESIAN_POINT ( 'NONE',  ( -113.7382910024855533, -286.0177996698006950, -267.1573561207084140 ) ) ;
#12863=CARTESIAN_POINT ( 'NONE',  ( -69.19529939205334301, -282.2757161854602828, -336.4997186565072980 ) ) ;
#12864=CARTESIAN_POINT ( 'NONE',  ( -52.24914702988790793, -281.8615825267725654, -196.8044388012513366 ) ) ;
#12865=CARTESIAN_POINT ( 'NONE',  ( -7.692542024774548182, -274.5967035126004134, -199.2416801386512759 ) ) ;
#12866=CARTESIAN_POINT ( 'NONE',  ( 22.75968331239080911, -274.7405064548540281, -222.2068134651589162 ) ) ;
#12867=CARTESIAN_POINT ( 'NONE',  ( -109.9920108096132907, -298.2624124991974099, -286.5859927051400291 ) ) ;
#12871=CARTESIAN_POINT ( 'NONE',  ( -109.1821406003631978, -294.3837371573162613, -294.4288680343846636 ) ) ;
#12872=CARTESIAN_POINT ( 'NONE',  ( 33.64483044088866137, -275.2883494617894939, -287.7025516250984651 ) ) ;
#12873=CARTESIAN_POINT ( 'NONE',  ( -57.69426220730361621, -287.5460253404503419, -199.1477575376319464 ) ) ;
#12875=CARTESIAN_POINT ( 'NONE',  ( -1.018999310745072329, -296.0991715007161247, -337.4830177702351079 ) ) ;
#12876=CARTESIAN_POINT ( 'NONE',  ( -16.59956865210886434, -295.9951589218848653, -344.1573245609079663 ) ) ;
#12877=CARTESIAN_POINT ( 'NONE',  ( -98.84141721499349842, -291.9725364720823109, -313.0194412108830306 ) ) ;
#12878=CARTESIAN_POINT ( 'NONE',  ( -109.7399485568272723, -276.7964472466167081, -251.3761731370418602 ) ) ;
#12879=CARTESIAN_POINT ( 'NONE',  ( -100.7060863049831028, -281.0017155072604282, -231.1952410859327358 ) ) ;
#12880=CARTESIAN_POINT ( 'NONE',  ( -70.38483200865748302, -293.5710378368185047, -337.0654329635964928 ) ) ;
#12881=CARTESIAN_POINT ( 'NONE',  ( -78.46902979880994167, -285.4598642992408486, -333.9916785110635260 ) ) ;
#12883=CARTESIAN_POINT ( 'NONE',  ( -103.7597201120072583, -283.8911662319997617, -239.2106381586119142 ) ) ;
#12884=CARTESIAN_POINT ( 'NONE',  ( 46.98483951095349909, 11.15615824186278005, -331.1643732653742518 ) ) ;
#12886=CARTESIAN_POINT ( 'NONE',  ( -102.2552504324740994, -284.6733491823260351, -236.9198489641671301 ) ) ;
#12888=CARTESIAN_POINT ( 'NONE',  ( -3.018798571468261471, -283.6890445247593675, -338.9572776022216658 ) ) ;
#12889=CARTESIAN_POINT ( 'NONE',  ( -108.6531869413102811, -283.7051868586116257, -242.2405080801414670 ) ) ;
#12890=CARTESIAN_POINT ( 'NONE',  ( -103.2158630380051534, -280.0100581557256874, -230.8443507147514993 ) ) ;
#12892=CARTESIAN_POINT ( 'NONE',  ( -112.6120434078924575, -279.9140996689043845, -282.8944007058090051 ) ) ;
#12893=CARTESIAN_POINT ( 'NONE',  ( -8.906525419621885931, -281.0659159457808869, -198.9135594103130416 ) ) ;
#12894=CARTESIAN_POINT ( 'NONE',  ( -53.35057174420112602, -274.7666405000204009, -340.3538533559490702 ) ) ;
#12895=CARTESIAN_POINT ( 'NONE',  ( 175.2421902450908533, 242.6932815909999306, -179.6955966096621466 ) ) ;
#12896=EDGE_LOOP ( 'NONE', ( #75994, #73754, #68849, #92774 ) ) ;
#12897=CARTESIAN_POINT ( 'NONE',  ( -36.74644463627333835, -276.0598066089866052, -195.5174214593769193 ) ) ;
#12898=CARTESIAN_POINT ( 'NONE',  ( 44.42952696178269179, 12.78217976624798879, -331.7054304614241005 ) ) ;
#12899=CARTESIAN_POINT ( 'NONE',  ( -77.69020372323333845, -277.5280634081740914, -207.4994738444986808 ) ) ;
#12900=CARTESIAN_POINT ( 'NONE',  ( -11.51897694432051900, -294.1439391656043085, -198.8414213500067547 ) ) ;
#12901=CARTESIAN_POINT ( 'NONE',  ( -69.77674570138822219, -294.8395733358574944, -335.8734106245736939 ) ) ;
#12902=CARTESIAN_POINT ( 'NONE',  ( -108.7436840526381587, -289.6958211182744094, -299.0191638811032817 ) ) ;
#12903=CARTESIAN_POINT ( 'NONE',  ( -68.00650040173375999, -294.0216715123015661, -340.3488048878853078 ) ) ;
#12904=CARTESIAN_POINT ( 'NONE',  ( -65.37846775173028391, -284.0794418382948834, -202.0397517839834052 ) ) ;
#12905=CARTESIAN_POINT ( 'NONE',  ( -103.5212993092666096, -292.8630687204117748, -236.6150369288597233 ) ) ;
#12906=CARTESIAN_POINT ( 'NONE',  ( -11.76335267563215758, -284.8712125508853887, -201.2492095016121993 ) ) ;
#12907=CARTESIAN_POINT ( 'NONE',  ( -83.08869381652628761, -285.0083970499785551, -327.9455883539226306 ) ) ;
#12909=CARTESIAN_POINT ( 'NONE',  ( -77.05782195959486103, -292.4753047542684499, -204.6077246947470485 ) ) ;
#12910=CARTESIAN_POINT ( 'NONE',  ( -34.83815681930158803, -283.5122410187837545, -343.3921976036638171 ) ) ;
#12911=CARTESIAN_POINT ( 'NONE',  ( -113.3787734148549617, -295.4639119296739977, -261.0674532495754647 ) ) ;
#12912=CARTESIAN_POINT ( 'NONE',  ( -108.6448071687833306, -290.9907923289092082, -298.9972096576212834 ) ) ;
#12913=CARTESIAN_POINT ( 'NONE',  ( -71.87322625413527533, -289.9887247457808144, -339.1150313759645769 ) ) ;
#12914=CARTESIAN_POINT ( 'NONE',  ( 17.77479428399139749, -287.0364495593480001, -222.4949289944469797 ) ) ;
#12917=CARTESIAN_POINT ( 'NONE',  ( -94.63171407982453331, -297.7318221147525605, -319.9409504139586602 ) ) ;
#12918=CARTESIAN_POINT ( 'NONE',  ( -110.3375233717847550, -295.5287121118184928, -247.2747539743806158 ) ) ;
#12919=CARTESIAN_POINT ( 'NONE',  ( -19.46555647645083553, -279.3463875274569546, -199.2885757961579429 ) ) ;
#12920=CARTESIAN_POINT ( 'NONE',  ( 28.45317866480812086, -274.5376530778539177, -230.3774195733493855 ) ) ;
#12921=CARTESIAN_POINT ( 'NONE',  ( -104.5770583508462153, -294.6280095406722808, -300.6540327414994067 ) ) ;
#12922=CARTESIAN_POINT ( 'NONE',  ( 19.98044599088153817, -277.9663116656553257, -317.2014515432399548 ) ) ;
#12923=CARTESIAN_POINT ( 'NONE',  ( -79.53803314091729249, -271.6154073949409167, -209.2222210029422058 ) ) ;
#12924=CARTESIAN_POINT ( 'NONE',  ( -23.42860723102124254, -296.0755340508383711, -342.4793376116002150 ) ) ;
#12925=CARTESIAN_POINT ( 'NONE',  ( -6.622910189156639760, -295.7186998073491395, -336.9237352633185765 ) ) ;
#12927=CARTESIAN_POINT ( 'NONE',  ( -44.69789722621516859, -296.7437646801308802, -346.2580642009152712 ) ) ;
#12929=CARTESIAN_POINT ( 'NONE',  ( -33.42740386265555941, -296.1008865582589920, -195.1957734180984119 ) ) ;
#12930=CARTESIAN_POINT ( 'NONE',  ( -83.90032894964507193, -292.0440802214554878, -214.0034499143460778 ) ) ;
#12931=CARTESIAN_POINT ( 'NONE',  ( -31.28301405184805972, -274.9296399455838014, -193.7485750489041720 ) ) ;
#12932=CARTESIAN_POINT ( 'NONE',  ( -98.61123969104716025, -288.5653390216393177, -311.1445675930501693 ) ) ;
#12934=CARTESIAN_POINT ( 'NONE',  ( -46.87958923498909058, -274.4264582998733886, -194.0161405805469030 ) ) ;
#12935=CARTESIAN_POINT ( 'NONE',  ( -102.7852251685376785, -296.4450991252521703, -302.8672277728502422 ) ) ;
#12936=CARTESIAN_POINT ( 'NONE',  ( 26.44532598430231829, -282.9940970792346775, -230.1432839529457794 ) ) ;
#12937=CARTESIAN_POINT ( 'NONE',  ( 18.80967482594860130, -279.5246084189157045, -218.3965015245213408 ) ) ;
#12938=ADVANCED_FACE ( 'NONE', ( #34587 ), #33864, .F. ) ;
#12939=CARTESIAN_POINT ( 'NONE',  ( -54.11710349943030707, -276.6105596820148662, -345.4616639157244435 ) ) ;
#12940=CARTESIAN_POINT ( 'NONE',  ( 38.91001426787408235, -279.9468928874801463, -269.9550827114948106 ) ) ;
#12941=CARTESIAN_POINT ( 'NONE',  ( 26.31271014087302262, -279.0146858653869799, -230.2867233043065198 ) ) ;
#12943=CARTESIAN_POINT ( 'NONE',  ( -31.27317142014541318, -272.7049893050045739, -197.0097824073637582 ) ) ;
#12944=CARTESIAN_POINT ( 'NONE',  ( -112.2832128605261772, -280.5002450324488450, -274.4165853928661818 ) ) ;
#12945=CARTESIAN_POINT ( 'NONE',  ( 82.12347693879148380, -301.5478687382300222, -195.3203844934047311 ) ) ;
#12947=CARTESIAN_POINT ( 'NONE',  ( -35.47996997805969954, -296.3150216663414085, -194.3749935974277037 ) ) ;
#12948=CARTESIAN_POINT ( 'NONE',  ( -47.49624196822620092, -289.9439384386781740, -195.6405958643876204 ) ) ;
#12949=CARTESIAN_POINT ( 'NONE',  ( -64.38880357372521246, -291.7088732485124183, -198.2115734829788494 ) ) ;
#12950=CARTESIAN_POINT ( 'NONE',  ( 37.31975202022893967, -277.6693848268944862, -279.4991216609959679 ) ) ;
#12951=CARTESIAN_POINT ( 'NONE',  ( 4.054503818188253561, -272.6092366707648580, -207.7582114533805111 ) ) ;
#12953=CARTESIAN_POINT ( 'NONE',  ( -19.23923631631214448, -284.7412941686194472, -343.7745435736915169 ) ) ;
#12955=CARTESIAN_POINT ( 'NONE',  ( -9.014712081650293030, -284.4224206629857008, -200.9026544543546322 ) ) ;
#12957=CARTESIAN_POINT ( 'NONE',  ( 23.25216914410762215, -292.9213619464269414, -311.8687276326587039 ) ) ;
#12958=CARTESIAN_POINT ( 'NONE',  ( -5.243467808546058428, -284.6186346517775405, -203.4100468069346164 ) ) ;
#12959=CARTESIAN_POINT ( 'NONE',  ( 19.47122598114649961, -292.2309370901153329, -319.3428406447990824 ) ) ;
#12960=CARTESIAN_POINT ( 'NONE',  ( -41.55043331426213626, -281.5839976357776209, -346.6034860639621797 ) ) ;
#12961=CARTESIAN_POINT ( 'NONE',  ( -108.7517935008075085, -280.3961540006297923, -251.6824428764662400 ) ) ;
#12962=CARTESIAN_POINT ( 'NONE',  ( 38.16286399629263570, -288.5937650722264607, -257.3585025162579427 ) ) ;
#12963=CARTESIAN_POINT ( 'NONE',  ( 33.63291808743266387, -280.1402041058048553, -297.5010807902614829 ) ) ;
#12964=CARTESIAN_POINT ( 'NONE',  ( -2.186385233618647117, -286.5309173464250989, -206.3270319700781386 ) ) ;
#12965=CARTESIAN_POINT ( 'NONE',  ( -77.15578709489253129, -280.9326792680672611, -208.4116458274089894 ) ) ;
#12966=CARTESIAN_POINT ( 'NONE',  ( 25.26919453014395245, -281.8339834524051639, -232.4148785957278847 ) ) ;
#12967=CARTESIAN_POINT ( 'NONE',  ( -75.30046551474629268, -287.5290830154123682, -205.2046368264381329 ) ) ;
#12969=CARTESIAN_POINT ( 'NONE',  ( -99.09116807551103534, -296.9975421848020005, -224.3390779066832863 ) ) ;
#12970=CARTESIAN_POINT ( 'NONE',  ( -103.8870829031500591, -292.9825257437038886, -236.4300764022034684 ) ) ;
#12973=CARTESIAN_POINT ( 'NONE',  ( -88.47809603358389552, -298.1948066931273615, -334.5364918783848793 ) ) ;
#12975=CARTESIAN_POINT ( 'NONE',  ( -49.39943109210859973, -271.8987596746026156, -196.1153375487108690 ) ) ;
#12976=CARTESIAN_POINT ( 'NONE',  ( -79.05622870561278148, -294.0045880868150334, -334.1289666190540402 ) ) ;
#12977=CARTESIAN_POINT ( 'NONE',  ( -66.83843959832350379, -297.1625678877363157, -203.5048449782682951 ) ) ;
#12978=CARTESIAN_POINT ( 'NONE',  ( 20.91739395978089888, -289.7020571447915813, -315.5101034797131661 ) ) ;
#12979=CARTESIAN_POINT ( 'NONE',  ( 33.94136413198724256, -283.5719364506622355, -290.2784161074279154 ) ) ;
#12980=CARTESIAN_POINT ( 'NONE',  ( -98.54619287633666147, -291.3638534986807826, -316.1278726033087310 ) ) ;
#12981=CARTESIAN_POINT ( 'NONE',  ( -106.0631321381372345, -291.4313685608193509, -304.1068196155210330 ) ) ;
#12982=CARTESIAN_POINT ( 'NONE',  ( -60.62300076900870494, -287.7502956331037467, -199.0660852843546138 ) ) ;
#12983=CARTESIAN_POINT ( 'NONE',  ( -6.232313260442182923, -280.6163704206869625, -199.9110166355659999 ) ) ;
#12984=CARTESIAN_POINT ( 'NONE',  ( 12.42859662767392059, -292.4455311813479170, -327.2831899499475981 ) ) ;
#12985=CARTESIAN_POINT ( 'NONE',  ( 25.92911623498276441, -281.9654566476276614, -314.2682874409046008 ) ) ;
#12986=CARTESIAN_POINT ( 'NONE',  ( -8.512653817610086548, -276.2938300422520683, -201.8975937578110802 ) ) ;
#12987=CARTESIAN_POINT ( 'NONE',  ( -53.35057174420112602, -282.3376638359844151, -200.3683826091709648 ) ) ;
#12988=CARTESIAN_POINT ( 'NONE',  ( 25.21966653337349840, -274.3700642518234645, -313.5804427869251185 ) ) ;
#12990=CARTESIAN_POINT ( 'NONE',  ( 34.12670680731089590, -280.8590426642495004, -255.1273190691508717 ) ) ;
#12991=CARTESIAN_POINT ( 'NONE',  ( -95.83599969088056980, -279.0871572331816424, -319.8427136825275738 ) ) ;
#12992=CARTESIAN_POINT ( 'NONE',  ( -38.10416821729442205, -275.3575766837120113, -196.8719206675939120 ) ) ;
#12993=CARTESIAN_POINT ( 'NONE',  ( -18.22898541540989115, -285.3512484480527860, -195.9588593539383794 ) ) ;
#12994=CARTESIAN_POINT ( 'NONE',  ( -107.9115756068716934, -292.0185642881020271, -292.8433918286247604 ) ) ;
#12995=CARTESIAN_POINT ( 'NONE',  ( -107.3506509167288385, -274.5410603450831104, -240.1412642514910374 ) ) ;
#12997=CARTESIAN_POINT ( 'NONE',  ( -94.72774099892640720, -274.5568185179035368, -219.7632861451976964 ) ) ;
#12999=CARTESIAN_POINT ( 'NONE',  ( -5.067995457303488216, -276.4484191422664594, -335.8533099289364259 ) ) ;
#13001=CARTESIAN_POINT ( 'NONE',  ( -83.47038087616263624, -297.6859669677472198, -329.3523175785386456 ) ) ;
#13002=CARTESIAN_POINT ( 'NONE',  ( -95.53196003705915018, -283.2013669065388513, -223.2884845940816660 ) ) ;
#13003=CARTESIAN_POINT ( 'NONE',  ( 39.63502101225977015, -293.1823495328365539, -267.4416400126836493 ) ) ;
#13004=CARTESIAN_POINT ( 'NONE',  ( 18.65273970250616387, -274.2618134532861518, -319.7409997881770778 ) ) ;
#13005=CARTESIAN_POINT ( 'NONE',  ( 38.83979864417077721, -289.1310588803307269, -268.6819341795176683 ) ) ;
#13006=CARTESIAN_POINT ( 'NONE',  ( -81.90610081340983584, -290.3491984532741981, -212.0882981895577188 ) ) ;
#13008=CARTESIAN_POINT ( 'NONE',  ( -68.07498969488386820, -290.2312129412768513, -200.3892241402413958 ) ) ;
#13009=CARTESIAN_POINT ( 'NONE',  ( -89.82856992196482793, -290.9522623577512377, -219.5948300937954514 ) ) ;
#13011=CARTESIAN_POINT ( 'NONE',  ( 29.85406381361815775, -288.1499330768536424, -233.2885271821867263 ) ) ;
#13012=CARTESIAN_POINT ( 'NONE',  ( -106.2827641536922272, -278.5635628395485810, -294.5813718221854742 ) ) ;
#13013=CARTESIAN_POINT ( 'NONE',  ( -30.63174672532532483, -293.8895191435576635, -346.7579047930188381 ) ) ;
#13014=CARTESIAN_POINT ( 'NONE',  ( -110.5859223994486626, -284.9082078208705298, -293.8266679287471561 ) ) ;
#13015=CARTESIAN_POINT ( 'NONE',  ( -106.9847104616108169, -284.4652246864134213, -303.1573891596178782 ) ) ;
#13016=CARTESIAN_POINT ( 'NONE',  ( -7.240884720463841795, -282.9794092498300984, -336.9032389114767057 ) ) ;
#13017=CARTESIAN_POINT ( 'NONE',  ( 25.45548143946952280, -22.91915814266209139, -345.1898414876856123 ) ) ;
#13018=CARTESIAN_POINT ( 'NONE',  ( -84.98129659660571633, -218.6007500822886698, -351.5046871484345274 ) ) ;
#13019=CARTESIAN_POINT ( 'NONE',  ( -111.8582150891662650, -270.5933945666634486, -270.3361783062999848 ) ) ;
#13020=CARTESIAN_POINT ( 'NONE',  ( 33.39571117036256709, -274.9953942226081836, -289.0378513739431696 ) ) ;
#13021=CARTESIAN_POINT ( 'NONE',  ( 20.93559475271237957, -273.8494510930563024, -225.8659299357156272 ) ) ;
#13022=CARTESIAN_POINT ( 'NONE',  ( -104.5522034484624356, -295.5727186817607048, -307.9170098336240926 ) ) ;
#13023=CARTESIAN_POINT ( 'NONE',  ( 197.5414458789393279, 281.6342289571271635, -110.4094420167315747 ) ) ;
#13024=CARTESIAN_POINT ( 'NONE',  ( 38.64572984594678218, -274.3545847953408270, -279.7044014839854640 ) ) ;
#13025=CARTESIAN_POINT ( 'NONE',  ( -109.3792446928450062, -298.6458408137543188, -252.3797673348543356 ) ) ;
#13026=CARTESIAN_POINT ( 'NONE',  ( -90.99475429689738348, -292.3472438696775271, -220.3868148038729942 ) ) ;
#13028=CARTESIAN_POINT ( 'NONE',  ( -113.8872091155850086, -297.5744272293689505, -263.9022236224023459 ) ) ;
#13030=CARTESIAN_POINT ( 'NONE',  ( -29.16001087379421008, -289.4380187972297449, -342.9631041988759534 ) ) ;
#13031=CARTESIAN_POINT ( 'NONE',  ( -104.4568706530885862, -296.8676899480395264, -307.8825977626626695 ) ) ;
#13032=CARTESIAN_POINT ( 'NONE',  ( -13.79491257405529936, -295.2468845651835636, -343.6077950334290563 ) ) ;
#13033=CARTESIAN_POINT ( 'NONE',  ( 33.94934584891574758, -293.5109205467754805, -254.6002432636048525 ) ) ;
#13035=CARTESIAN_POINT ( 'NONE',  ( 23.22826953505513004, -278.0846408482625520, -315.5340410194270362 ) ) ;
#13036=CARTESIAN_POINT ( 'NONE',  ( 34.26944720202351391, -280.7012568199019711, -242.0843685209363798 ) ) ;
#13037=CARTESIAN_POINT ( 'NONE',  ( 33.47276509706586722, -276.7391968001456917, -289.0351631674133728 ) ) ;
#13038=CARTESIAN_POINT ( 'NONE',  ( 19.26578590883388031, -276.6148802463860648, -219.5929287616562249 ) ) ;
#13039=CARTESIAN_POINT ( 'NONE',  ( -34.38149873138987545, -275.0352162665833475, -345.6581565222509766 ) ) ;
#13040=CARTESIAN_POINT ( 'NONE',  ( -110.1526375655736416, -297.2966128626596287, -263.2980455959078654 ) ) ;
#13041=CARTESIAN_POINT ( 'NONE',  ( -71.21807424455170121, -294.0831976299256212, -335.7033590814297668 ) ) ;
#13043=CARTESIAN_POINT ( 'NONE',  ( -114.1497829663616272, -279.1005366207717771, -265.8839186587057384 ) ) ;
#13044=CARTESIAN_POINT ( 'NONE',  ( 30.27882968814611075, -276.0888587007171964, -297.9995209854804443 ) ) ;
#13045=CARTESIAN_POINT ( 'NONE',  ( -23.85626398058290221, -284.9056691563109780, -194.9982742528010817 ) ) ;
#13046=CARTESIAN_POINT ( 'NONE',  ( -64.89429579173447848, -299.6934189820075289, -200.3706295696523512 ) ) ;
#13048=CARTESIAN_POINT ( 'NONE',  ( 35.84217703549991541, -286.7224235668668371, -268.3181286021995788 ) ) ;
#13049=CARTESIAN_POINT ( 'NONE',  ( -88.21104146923185851, -277.5683815971250965, -216.5289483050232207 ) ) ;
#13050=CARTESIAN_POINT ( 'NONE',  ( -106.9966160351694384, -277.4416931496293159, -246.4651712220571653 ) ) ;
#13051=CARTESIAN_POINT ( 'NONE',  ( -87.92492737254799806, -281.8453857191601060, -325.0453156086622926 ) ) ;
#13053=CARTESIAN_POINT ( 'NONE',  ( -41.52575460317072498, -287.9996389986643521, -195.4652721004907789 ) ) ;
#13054=CARTESIAN_POINT ( 'NONE',  ( -73.02167804767384496, -278.7412739595085895, -334.5165905436804792 ) ) ;
#13056=CARTESIAN_POINT ( 'NONE',  ( 21.52209751963951945, -294.9138446577944137, -223.8642244884936474 ) ) ;
#13057=CARTESIAN_POINT ( 'NONE',  ( -94.46403227200600838, -276.1049076941987437, -320.4711288144811192 ) ) ;
#13058=CARTESIAN_POINT ( 'NONE',  ( 32.15613502198027618, -275.9012243513387261, -247.5280129497101598 ) ) ;
#13059=CARTESIAN_POINT ( 'NONE',  ( 5.891857655372181313, -284.4680844835685321, -331.9137060373463441 ) ) ;
#13061=CARTESIAN_POINT ( 'NONE',  ( 30.40733201666325414, -289.9117772095127066, -303.9363763766240254 ) ) ;
#13062=CARTESIAN_POINT ( 'NONE',  ( -99.37396939430259124, -295.1236747451754354, -228.1168886516929035 ) ) ;
#13064=CARTESIAN_POINT ( 'NONE',  ( 11.88921313126211565, -273.4378169972527530, -215.7255500305664100 ) ) ;
#13065=CARTESIAN_POINT ( 'NONE',  ( -25.18384741761302337, -290.3482310621494662, -197.0759035933843393 ) ) ;
#13066=CARTESIAN_POINT ( 'NONE',  ( 138.4517698930976621, 181.0451598467585939, -241.7086681466011271 ) ) ;
#13068=CARTESIAN_POINT ( 'NONE',  ( -113.4946700605296286, -289.0931220403244311, -265.5203616729537544 ) ) ;
#13069=CARTESIAN_POINT ( 'NONE',  ( -109.4979902225110351, -285.9493890096130713, -285.9100982614749569 ) ) ;
#13070=CARTESIAN_POINT ( 'NONE',  ( 32.93096371817990331, -285.4181899331740624, -241.3146186784875340 ) ) ;
#13071=CARTESIAN_POINT ( 'NONE',  ( -69.04509906562462618, -287.0520909847288635, -203.9373558796297914 ) ) ;
#13072=CARTESIAN_POINT ( 'NONE',  ( -33.23980564483053257, -286.9078165065594135, -197.2647899026690936 ) ) ;
#13073=CARTESIAN_POINT ( 'NONE',  ( -73.90340961557159005, -293.5488941257589772, -204.4699334168999769 ) ) ;
#13074=CARTESIAN_POINT ( 'NONE',  ( 13.88854926926081212, -274.4205738416655436, -325.9730657272613712 ) ) ;
#13075=CARTESIAN_POINT ( 'NONE',  ( 28.48226406185101567, -275.3631484397516260, -230.3474458447223299 ) ) ;
#13076=CARTESIAN_POINT ( 'NONE',  ( -112.5706509030317903, -288.7289087283336926, -262.7570976468396680 ) ) ;
#13077=CARTESIAN_POINT ( 'NONE',  ( -34.29109513770518447, -277.0147884556819236, -347.3006644407546446 ) ) ;
#13078=CARTESIAN_POINT ( 'NONE',  ( -64.13638638193125985, -297.3831825584928765, -340.0857498392702496 ) ) ;
#13081=CARTESIAN_POINT ( 'NONE',  ( -96.32749537631258363, -282.6262012106118391, -314.2008196018245485 ) ) ;
#13082=CARTESIAN_POINT ( 'NONE',  ( -74.00735558725403962, -277.5648361339606254, -204.9345915605718460 ) ) ;
#13084=CARTESIAN_POINT ( 'NONE',  ( -36.92391245623485929, -272.5372109556587361, -194.0426576421041318 ) ) ;
#13085=CARTESIAN_POINT ( 'NONE',  ( -56.63505139962715873, -276.6559627413939211, -340.9236851857388046 ) ) ;
#13086=CARTESIAN_POINT ( 'NONE',  ( 35.52649840252095714, -295.2203273087150706, -281.6905790513746979 ) ) ;
#13087=CARTESIAN_POINT ( 'NONE',  ( 31.74898901914198390, -280.0423713706244939, -236.9527273951630661 ) ) ;
#13088=CARTESIAN_POINT ( 'NONE',  ( -97.36938833928104486, -296.9102845637692667, -312.3144861001824211 ) ) ;
#13089=CARTESIAN_POINT ( 'NONE',  ( -41.89933291420142325, -296.4234854456285575, -346.7841541728756170 ) ) ;
#13090=CARTESIAN_POINT ( 'NONE',  ( -96.09905745091680274, -296.9928507279720975, -227.0205856304320662 ) ) ;
#13091=CARTESIAN_POINT ( 'NONE',  ( -105.3811154459989439, -292.9668639513399739, -238.8073763842450603 ) ) ;
#13092=CARTESIAN_POINT ( 'NONE',  ( -85.51456223545741864, -285.5733461173820729, -210.2913638556467788 ) ) ;
#13093=CARTESIAN_POINT ( 'NONE',  ( -100.1707604848266300, -271.2597680969976182, -227.9261168779661659 ) ) ;
#13094=CARTESIAN_POINT ( 'NONE',  ( -73.17575076540566670, -289.3471611511228616, -338.5295305579006140 ) ) ;
#13095=CARTESIAN_POINT ( 'NONE',  ( -82.29815515474960819, -281.4155730172693097, -210.7079116666343452 ) ) ;
#13096=CARTESIAN_POINT ( 'NONE',  ( -42.67935526091009990, -285.0419367525855705, -197.3079294672511139 ) ) ;
#13097=CARTESIAN_POINT ( 'NONE',  ( -71.03151128435941075, -287.4966203679318255, -337.3685599341721399 ) ) ;
#13098=CARTESIAN_POINT ( 'NONE',  ( -30.04969936926732288, -125.9919632799748683, -361.3284013991797110 ) ) ;
#13099=CARTESIAN_POINT ( 'NONE',  ( 13.18663659086080031, -286.2891020732555489, -217.5193923262981457 ) ) ;
#13101=CARTESIAN_POINT ( 'NONE',  ( -55.63446246692085850, -284.2232996921275685, -344.9144214526192513 ) ) ;
#13102=CARTESIAN_POINT ( 'NONE',  ( -111.6971304372364813, -289.3707883968131114, -289.4948841157578272 ) ) ;
#13103=CARTESIAN_POINT ( 'NONE',  ( -110.9634365019315823, -280.4015158755510697, -250.6566750267772932 ) ) ;
#13105=CARTESIAN_POINT ( 'NONE',  ( -105.7422402517998421, -280.3123565708022511, -235.9696995371090225 ) ) ;
#13106=CARTESIAN_POINT ( 'NONE',  ( 34.56745690993932385, -281.2196164527435371, -257.7884039319196177 ) ) ;
#13107=CARTESIAN_POINT ( 'NONE',  ( 25.45452036444216759, -276.9991902721627071, -229.3533706632188682 ) ) ;
#13108=CARTESIAN_POINT ( 'NONE',  ( -64.26618685996827196, -295.3939646809603801, -342.5003723051854649 ) ) ;
#13109=CARTESIAN_POINT ( 'NONE',  ( -111.9820258855963573, -288.5617055105353757, -271.1787795172390361 ) ) ;
#13110=CARTESIAN_POINT ( 'NONE',  ( -75.83200796478132588, -294.4991503684483973, -332.8119906804576544 ) ) ;
#13113=CARTESIAN_POINT ( 'NONE',  ( -32.01880167513055397, -284.9046274631432993, -344.6105688262024955 ) ) ;
#13114=CARTESIAN_POINT ( 'NONE',  ( -110.0709601562335109, -296.3120770961277799, -263.2933892711366752 ) ) ;
#13115=CARTESIAN_POINT ( 'NONE',  ( 29.20058581790802421, -294.1344513205390285, -232.2347925612275787 ) ) ;
#13116=CARTESIAN_POINT ( 'NONE',  ( -91.73535024486200484, -284.5053536241732104, -319.2187010217430725 ) ) ;
#13117=CARTESIAN_POINT ( 'NONE',  ( 25.14237595999650310, -274.0181648292290788, -225.7453482768341644 ) ) ;
#13118=CARTESIAN_POINT ( 'NONE',  ( -113.5662411612886302, -291.3356247030081363, -259.8155710765743152 ) ) ;
#13119=CARTESIAN_POINT ( 'NONE',  ( -112.2623025429352595, -282.8394819047600777, -258.7371879021617929 ) ) ;
#13120=CARTESIAN_POINT ( 'NONE',  ( -97.44971819883089381, -291.5297832156729214, -222.2698458504537484 ) ) ;
#13121=CARTESIAN_POINT ( 'NONE',  ( 21.98134771310451896, -288.4804618505643248, -312.9388525589154710 ) ) ;
#13124=CARTESIAN_POINT ( 'NONE',  ( -107.5458925959985947, -264.4132577019892665, -305.3929582931264122 ) ) ;
#13125=CARTESIAN_POINT ( 'NONE',  ( -24.62984935714912282, -284.4130276570701312, -345.6551408998312240 ) ) ;
#13126=CARTESIAN_POINT ( 'NONE',  ( -20.25526795762938548, -286.3380690714490697, -345.3683826091709648 ) ) ;
#13128=CARTESIAN_POINT ( 'NONE',  ( -46.48142157134198982, -278.8539036382458107, -197.5726601185043307 ) ) ;
#13129=CARTESIAN_POINT ( 'NONE',  ( -65.09141310736701769, -277.0715631795633840, -342.2205774995742900 ) ) ;
#13130=CARTESIAN_POINT ( 'NONE',  ( -59.71956267270761032, -279.3428711032244678, -341.7702188895860900 ) ) ;
#13131=CARTESIAN_POINT ( 'NONE',  ( 46.92461508910208323, 10.64641740143134641, -329.6966147455941609 ) ) ;
#13132=CARTESIAN_POINT ( 'NONE',  ( 36.61688497611752524, -280.3690785119252382, -289.5635653221009420 ) ) ;
#13133=CARTESIAN_POINT ( 'NONE',  ( -111.0411660237937923, -282.7260753879510276, -258.4382146118613832 ) ) ;
#13134=CARTESIAN_POINT ( 'NONE',  ( -90.93689066507117502, -299.0640243673317400, -216.4952701389109961 ) ) ;
#13135=CARTESIAN_POINT ( 'NONE',  ( 1.607939867105836473, -295.0087424573893031, -332.2345811614868012 ) ) ;
#13137=CARTESIAN_POINT ( 'NONE',  ( -108.8340143552357944, -289.0137826064509454, -287.3932196156199552 ) ) ;
#13138=CARTESIAN_POINT ( 'NONE',  ( 22.67358366012044613, -275.5584672508655331, -222.2624020364694672 ) ) ;
#13139=CARTESIAN_POINT ( 'NONE',  ( -100.7177656438344826, -273.0497703128482385, -234.0313802245705119 ) ) ;
#13144=CARTESIAN_POINT ( 'NONE',  ( 36.01230307701023037, -282.6442167609558282, -271.3040711246267165 ) ) ;
#13145=CARTESIAN_POINT ( 'NONE',  ( -61.74371412948401172, -281.4996016295623917, -198.3437147946767425 ) ) ;
#13146=CARTESIAN_POINT ( 'NONE',  ( -45.67811780719655701, -282.2190079251647035, -343.1715554817286034 ) ) ;
#13147=CARTESIAN_POINT ( 'NONE',  ( -13.94161494949410773, -282.2192806148665909, -199.8560781612178516 ) ) ;
#13148=CARTESIAN_POINT ( 'NONE',  ( 24.55632538609000193, -274.5815952029155937, -310.4469483047266749 ) ) ;
#13151=CARTESIAN_POINT ( 'NONE',  ( -31.45241933482986596, -277.7825403288708230, -347.0261310258046592 ) ) ;
#13155=CARTESIAN_POINT ( 'NONE',  ( -80.59635609174226545, -285.6149197981504244, -332.1290540324805534 ) ) ;
#13156=CARTESIAN_POINT ( 'NONE',  ( 32.90235342443019562, -293.0198240527508915, -290.8603332812532472 ) ) ;
#13157=CARTESIAN_POINT ( 'NONE',  ( 39.50202748138706710, -286.9516424454297976, -274.4258296723526769 ) ) ;
#13158=CARTESIAN_POINT ( 'NONE',  ( -104.3941293239210069, -283.2108059009918861, -238.9036887440992700 ) ) ;
#13159=CARTESIAN_POINT ( 'NONE',  ( -110.0836111539618827, -282.9768764429899761, -281.8236110394187790 ) ) ;
#13160=CARTESIAN_POINT ( 'NONE',  ( -72.86463856696799724, -287.7694792911642026, -335.2925807679086461 ) ) ;
#13161=CARTESIAN_POINT ( 'NONE',  ( 24.47309893579775775, -283.3028150041392905, -310.0280693981140416 ) ) ;
#13162=CARTESIAN_POINT ( 'NONE',  ( 35.35315640183767982, -273.3149533290148270, -251.9096008031456790 ) ) ;
#13163=CARTESIAN_POINT ( 'NONE',  ( 26.47897666945932471, -285.3993546640204499, -228.7274581860868068 ) ) ;
#13164=CARTESIAN_POINT ( 'NONE',  ( -54.17178713204996399, -299.8361736930494885, -197.2738494807453264 ) ) ;
#13165=CARTESIAN_POINT ( 'NONE',  ( -110.5678219994499614, -282.7694014896367776, -253.3916304481684278 ) ) ;
#13166=CARTESIAN_POINT ( 'NONE',  ( -34.31556683640382488, -281.0323473273051604, -197.1757865294947862 ) ) ;
#13167=CARTESIAN_POINT ( 'NONE',  ( 37.80659957834622986, -289.5310266043937304, -268.6993494226722987 ) ) ;
#13170=CARTESIAN_POINT ( 'NONE',  ( -108.0806307988865598, -298.1282563709747819, -297.0664273263981272 ) ) ;
#13172=CARTESIAN_POINT ( 'NONE',  ( -98.53179750385400837, -275.9623592474047200, -313.7513081070798080 ) ) ;
#13173=CARTESIAN_POINT ( 'NONE',  ( -110.2743876131848424, -290.0562869382329154, -246.0082799058550904 ) ) ;
#13174=CARTESIAN_POINT ( 'NONE',  ( -20.68723561645209230, -293.2347711971108311, -342.3100293269384906 ) ) ;
#13175=CARTESIAN_POINT ( 'NONE',  ( -59.86897441637935202, -278.4390357109370484, -200.3520043454716131 ) ) ;
#13176=CARTESIAN_POINT ( 'NONE',  ( 97.23951108435230140, -297.8936950320585311, -196.1691743667933281 ) ) ;
#13177=CARTESIAN_POINT ( 'NONE',  ( 19.71814889672734949, -294.2161614112207531, -224.0225727172560539 ) ) ;
#13178=CARTESIAN_POINT ( 'NONE',  ( -95.99890600148557951, -287.6948066931273615, -223.6242672951989618 ) ) ;
#13179=CARTESIAN_POINT ( 'NONE',  ( -110.5556815663805565, -294.7593249774552078, -291.9112155208854915 ) ) ;
#13180=CARTESIAN_POINT ( 'NONE',  ( 12.71320640249439649, -289.9405463420261526, -324.6610746390530267 ) ) ;
#13182=CARTESIAN_POINT ( 'NONE',  ( 5.937709055172086359, -290.8701842108746405, -207.9041988101028835 ) ) ;
#13183=CARTESIAN_POINT ( 'NONE',  ( -85.05336978111068902, -291.1507612481433398, -326.4548881838513239 ) ) ;
#13185=CARTESIAN_POINT ( 'NONE',  ( -110.1345733825187096, -291.4515337883765369, -263.0263153193224070 ) ) ;
#13187=CARTESIAN_POINT ( 'NONE',  ( -103.4479646406618514, -291.2496717990660500, -309.1696249320678476 ) ) ;
#13188=CARTESIAN_POINT ( 'NONE',  ( 32.80281012903238747, -279.2139513374593207, -242.6839718336630654 ) ) ;
#13189=CARTESIAN_POINT ( 'NONE',  ( 33.64776568011784263, -293.3270417843093583, -253.2931411323557995 ) ) ;
#13190=CARTESIAN_POINT ( 'NONE',  ( 37.33125482342504142, -281.3170909118201166, -251.5741597718676417 ) ) ;
#13191=CARTESIAN_POINT ( 'NONE',  ( 37.31178805815597599, -280.9838636417387079, -251.5834452499970268 ) ) ;
#13192=CARTESIAN_POINT ( 'NONE',  ( -37.29173687890931888, -287.0513678794694670, -345.1944390038898973 ) ) ;
#13193=CARTESIAN_POINT ( 'NONE',  ( -6.766014609581612937, -280.7860669639875368, -338.0211470727738856 ) ) ;
#13194=CARTESIAN_POINT ( 'NONE',  ( -100.8120201606800634, -283.0891964045927125, -230.4046526402919426 ) ) ;
#13195=CARTESIAN_POINT ( 'NONE',  ( -14.41743743185335980, -278.8238259178663725, -197.5239472378277696 ) ) ;
#13196=CARTESIAN_POINT ( 'NONE',  ( -60.40381468904433859, -284.6803934060176857, -197.1645944589982093 ) ) ;
#13197=CARTESIAN_POINT ( 'NONE',  ( 22.40680990774804116, -275.7666686549721362, -228.1171986848795257 ) ) ;
#13199=CARTESIAN_POINT ( 'NONE',  ( 28.18763796841624369, -294.6956310842564903, -236.4148919517652985 ) ) ;
#13200=CARTESIAN_POINT ( 'NONE',  ( -7.934260883709791656, -275.8550925137372474, -199.7797254809386231 ) ) ;
#13201=CARTESIAN_POINT ( 'NONE',  ( -90.98626821953766353, -277.5068799541975295, -319.9760468343509388 ) ) ;
#13202=CARTESIAN_POINT ( 'NONE',  ( -70.89963077793883883, -291.7882434108544203, -201.0584102790545558 ) ) ;
#13203=CARTESIAN_POINT ( 'NONE',  ( -4.806455117229143426, -280.7069051779081406, -338.5719025573442309 ) ) ;
#13205=CARTESIAN_POINT ( 'NONE',  ( -110.5724608677903262, -289.6001785506539932, -271.1760589972295747 ) ) ;
#13206=CARTESIAN_POINT ( 'NONE',  ( -85.14078402382351385, -293.7120025835242814, -328.1559985897099523 ) ) ;
#13209=CARTESIAN_POINT ( 'NONE',  ( 23.39588687650400800, -292.4963591593925116, -229.7540500443035398 ) ) ;
#13211=CARTESIAN_POINT ( 'NONE',  ( -105.5795714935544112, -270.2666405000204009, -254.7536222014695397 ) ) ;
#13212=CARTESIAN_POINT ( 'NONE',  ( -102.1114193182946650, -296.1526308626056903, -229.1579180011978565 ) ) ;
#13213=CARTESIAN_POINT ( 'NONE',  ( 36.34147294759234370, -279.9165812688573283, -288.0542821122240866 ) ) ;
#13214=CARTESIAN_POINT ( 'NONE',  ( -91.56535843695301935, -286.6144295479914490, -216.3880399548188223 ) ) ;
#13215=CARTESIAN_POINT ( 'NONE',  ( 6.928609633152132297, -286.5069850563670002, -212.2529581264224419 ) ) ;
#13216=CARTESIAN_POINT ( 'NONE',  ( 34.84761650350014150, -277.2658398318063746, -285.1736234600069793 ) ) ;
#13217=CARTESIAN_POINT ( 'NONE',  ( -102.6415336746871674, -295.0556475122322695, -234.1978971791031370 ) ) ;
#13218=CARTESIAN_POINT ( 'NONE',  ( -108.5720322254002923, -298.0501579400387300, -290.4661870977500939 ) ) ;
#13219=CARTESIAN_POINT ( 'NONE',  ( 15.87527022550933431, -275.0718221360676807, -320.9089623607256954 ) ) ;
#13222=CARTESIAN_POINT ( 'NONE',  ( -113.5802273811413272, -296.3532992165808082, -259.6153921970017109 ) ) ;
#13223=CARTESIAN_POINT ( 'NONE',  ( 36.70431915697744074, -289.3733650648983371, -262.7125086578888045 ) ) ;
#13226=CARTESIAN_POINT ( 'NONE',  ( 35.22640332184441547, -288.3197350429695121, -279.1794528485765454 ) ) ;
#13228=CARTESIAN_POINT ( 'NONE',  ( -72.38866415002550525, -278.6586142101342602, -202.0491439790257857 ) ) ;
#13229=CARTESIAN_POINT ( 'NONE',  ( -84.11661706964751772, -296.3272961550989635, -331.4644670987712516 ) ) ;
#13230=CARTESIAN_POINT ( 'NONE',  ( -112.5897301300584985, -288.5739364756557848, -279.6292772476776349 ) ) ;
#13231=CARTESIAN_POINT ( 'NONE',  ( -105.9369329510236213, -296.4341113216348731, -305.4132990448233613 ) ) ;
#13232=CARTESIAN_POINT ( 'NONE',  ( 18.85208633331983563, -294.5465951587702875, -316.9909994963678059 ) ) ;
#13235=CARTESIAN_POINT ( 'NONE',  ( -69.05136874130262470, -290.9817495608907052, -339.7814949663526249 ) ) ;
#13236=CARTESIAN_POINT ( 'NONE',  ( 13.79469577742117714, -277.1948066931273047, -206.1857440867352693 ) ) ;
#13237=CARTESIAN_POINT ( 'NONE',  ( 26.63247633025644845, -281.4631305591855153, -313.0298129828989318 ) ) ;
#13238=CARTESIAN_POINT ( 'NONE',  ( 8.947493384365307278, -284.4160441842945488, -329.2264556882181523 ) ) ;
#13239=CARTESIAN_POINT ( 'NONE',  ( 0.01172085390532574128, -285.1138947430600297, -203.6878892655028892 ) ) ;
#13240=CARTESIAN_POINT ( 'NONE',  ( -100.9292277647859919, -289.1547526071266816, -231.6578813548579490 ) ) ;
#13241=CARTESIAN_POINT ( 'NONE',  ( 36.08224369344183913, -277.1749053330518677, -251.6734226417129321 ) ) ;
#13243=CARTESIAN_POINT ( 'NONE',  ( -106.4447276250628249, -278.8667357064120438, -246.6735348530797296 ) ) ;
#13244=CARTESIAN_POINT ( 'NONE',  ( 26.55194987874112300, -280.4158114208411234, -234.8435989714105006 ) ) ;
#13245=CARTESIAN_POINT ( 'NONE',  ( 20.59579138533102949, -277.3137119525053436, -320.6277849164667941 ) ) ;
#13246=CARTESIAN_POINT ( 'NONE',  ( -64.58667833182528284, -278.4993097295289886, -198.7110506695674701 ) ) ;
#13247=CARTESIAN_POINT ( 'NONE',  ( 177.9591486883064704, 253.1359646847975569, -165.0577554255288817 ) ) ;
#13248=CARTESIAN_POINT ( 'NONE',  ( -21.41534048864555473, -275.1928476423493635, -195.2667022053635151 ) ) ;
#13250=CARTESIAN_POINT ( 'NONE',  ( -107.4482365777889896, -274.4610668013719419, -240.0980019203336724 ) ) ;
#13251=CARTESIAN_POINT ( 'NONE',  ( -69.91165696735023971, -288.1233781216987495, -202.8022627189028810 ) ) ;
#13252=CARTESIAN_POINT ( 'NONE',  ( 82.61807361380685677, -301.9754278600166799, -194.6565851556404141 ) ) ;
#13253=CARTESIAN_POINT ( 'NONE',  ( 34.59012354649429710, -288.8184694851551626, -284.5695791274170006 ) ) ;
#13254=CARTESIAN_POINT ( 'NONE',  ( -104.5464866480762538, -286.7775138937134329, -234.7872787116800453 ) ) ;
#13255=CARTESIAN_POINT ( 'NONE',  ( 16.07979082962989636, -287.6181351154477284, -320.3354455872358244 ) ) ;
#13256=CARTESIAN_POINT ( 'NONE',  ( -100.9420828770734602, -284.6322877313541539, -226.9713096542522237 ) ) ;
#13257=CARTESIAN_POINT ( 'NONE',  ( -1.560555935284581475, -278.9347858037416472, -205.8153966966281132 ) ) ;
#13258=CARTESIAN_POINT ( 'NONE',  ( -16.85332721199014117, -288.1798577463021616, -198.9554921802975969 ) ) ;
#13259=CARTESIAN_POINT ( 'NONE',  ( 31.72684376296890818, -279.6908102532306657, -244.5194006846924424 ) ) ;
#13260=CARTESIAN_POINT ( 'NONE',  ( -93.08985695592467380, -279.1900557387588151, -318.2504329638941272 ) ) ;
#13261=CARTESIAN_POINT ( 'NONE',  ( 29.13944126306517646, -275.6348210317758571, -239.9361765859873685 ) ) ;
#13262=CARTESIAN_POINT ( 'NONE',  ( 32.49654814952607751, -286.7512063388230104, -301.8353581640465109 ) ) ;
#13263=CARTESIAN_POINT ( 'NONE',  ( -1.699944976556255982, -283.3948059126345811, -338.4333157630394453 ) ) ;
#13264=CARTESIAN_POINT ( 'NONE',  ( -110.6250167409816783, -284.7491674640791075, -293.8370608886457376 ) ) ;
#13265=CARTESIAN_POINT ( 'NONE',  ( 28.15200699728796252, -282.1571155903004069, -302.7182719269644053 ) ) ;
#13266=EDGE_LOOP ( 'NONE', ( #83894, #50637, #46520, #79412 ) ) ;
#13269=CARTESIAN_POINT ( 'NONE',  ( -79.82804075928844156, -291.4799941684432270, -333.1557867698357427 ) ) ;
#13270=CARTESIAN_POINT ( 'NONE',  ( -6.073065037973113256, -291.1393682624394614, -200.5216321678052509 ) ) ;
#13271=CARTESIAN_POINT ( 'NONE',  ( 9.067659185125956256, -297.8449062927535920, -197.2061706911376859 ) ) ;
#13272=CARTESIAN_POINT ( 'NONE',  ( 24.79900619645963644, -293.5030016537069741, -315.6805956289199457 ) ) ;
#13273=CARTESIAN_POINT ( 'NONE',  ( -61.50040692830693700, -287.8516458893056438, -339.9819815044450024 ) ) ;
#13274=CARTESIAN_POINT ( 'NONE',  ( 17.50396740551644825, -291.0890028363598390, -220.5875647013370724 ) ) ;
#13275=CARTESIAN_POINT ( 'NONE',  ( -110.7339212150326375, -291.7461608775428772, -271.2051485149819428 ) ) ;
#13277=CARTESIAN_POINT ( 'NONE',  ( -69.75114221688832572, -291.4789367044171513, -338.0112273654578985 ) ) ;
#13278=CARTESIAN_POINT ( 'NONE',  ( -83.12893142027415649, -289.4271986122948874, -210.6838080538360032 ) ) ;
#13279=CARTESIAN_POINT ( 'NONE',  ( -15.43824080252674413, -294.3356916071157912, -198.5771203424665146 ) ) ;
#13280=CARTESIAN_POINT ( 'NONE',  ( -60.06297201360979443, -286.6915577389756322, -200.7396252404172685 ) ) ;
#13281=CARTESIAN_POINT ( 'NONE',  ( 16.16620465187848765, -294.8088544805097513, -217.4964467051408974 ) ) ;
#13284=CARTESIAN_POINT ( 'NONE',  ( -34.19760693703548782, -276.0714005109367690, -195.0715338223843389 ) ) ;
#13285=CARTESIAN_POINT ( 'NONE',  ( -79.39714900560086619, -294.8017554348708131, -334.6689560731301754 ) ) ;
#13286=CARTESIAN_POINT ( 'NONE',  ( -40.80016292372313558, -272.2480494399781605, -196.3782366482245152 ) ) ;
#13287=CARTESIAN_POINT ( 'NONE',  ( -93.83512398945097743, -275.9552506792462623, -318.8359285611423388 ) ) ;
#13288=CARTESIAN_POINT ( 'NONE',  ( -35.81942213812178721, -299.3867755882932897, -196.8676142273301650 ) ) ;
#13289=CARTESIAN_POINT ( 'NONE',  ( 32.02582921031893193, -273.7123508140779222, -238.1920797287320397 ) ) ;
#13290=CARTESIAN_POINT ( 'NONE',  ( -72.38934847890529056, -296.9507956390861523, -335.0828205206771031 ) ) ;
#13292=CARTESIAN_POINT ( 'NONE',  ( -109.9634803927136346, -297.2329020091125926, -279.6364362873392793 ) ) ;
#13293=DIRECTION ( 'NONE',  ( -5.501794166262391869E-14, -0.01273136352371387336, 0.9999189529070978688 ) ) ;
#13294=CARTESIAN_POINT ( 'NONE',  ( 29.96425324400670931, -285.1267148682284756, -236.4743146447557933 ) ) ;
#13295=CARTESIAN_POINT ( 'NONE',  ( -71.90585480228867254, -273.4154427323843493, -206.0061226401631131 ) ) ;
#13296=CARTESIAN_POINT ( 'NONE',  ( -23.78590587996978911, -286.2206314835377725, -194.5095368467766264 ) ) ;
#13297=CARTESIAN_POINT ( 'NONE',  ( -96.37757304929139934, -289.5536556097736707, -319.7830831870003863 ) ) ;
#13298=CARTESIAN_POINT ( 'NONE',  ( -108.7782547143636265, -298.2234260206692511, -294.3449765333902519 ) ) ;
#13299=CARTESIAN_POINT ( 'NONE',  ( 2.525515051747646122, -292.5166364658471139, -333.7520399652273113 ) ) ;
#13300=CARTESIAN_POINT ( 'NONE',  ( -36.74352194544972150, -279.2566630304733621, -193.5119037040155945 ) ) ;
#13301=CARTESIAN_POINT ( 'NONE',  ( -110.4542110544635705, -282.2666405000204009, -253.6410175316879361 ) ) ;
#13303=CARTESIAN_POINT ( 'NONE',  ( -96.09535074574621660, -288.7327123666485136, -314.3723131753113762 ) ) ;
#13305=CARTESIAN_POINT ( 'NONE',  ( -48.37982755296233250, -287.1923466009893673, -344.5968286482300300 ) ) ;
#13306=CARTESIAN_POINT ( 'NONE',  ( -34.46092253694913410, -299.6889310377678726, -196.5603117501235033 ) ) ;
#13307=CARTESIAN_POINT ( 'NONE',  ( -14.42192968462125613, -281.7687458506202915, -197.4133293322394707 ) ) ;
#13308=CARTESIAN_POINT ( 'NONE',  ( -98.68457016061034892, -293.9788964776909097, -314.2150028641716517 ) ) ;
#13309=CARTESIAN_POINT ( 'NONE',  ( 33.65014977728414181, -281.7771729484286425, -287.4189228401804144 ) ) ;
#13310=CARTESIAN_POINT ( 'NONE',  ( -114.3661541337180125, -296.6924334952742583, -272.4719108930375455 ) ) ;
#13311=CARTESIAN_POINT ( 'NONE',  ( -110.9316044294118910, -274.0131273331129478, -267.6333776901211650 ) ) ;
#13312=CARTESIAN_POINT ( 'NONE',  ( 36.28629328887802785, -283.3689571366431323, -256.0810886769661465 ) ) ;
#13314=CARTESIAN_POINT ( 'NONE',  ( -102.9843626886730021, -295.1707710223560071, -302.9480397092364683 ) ) ;
#13316=CARTESIAN_POINT ( 'NONE',  ( -40.27429429716867304, -285.0690948919350376, -344.9482931299669417 ) ) ;
#13318=CARTESIAN_POINT ( 'NONE',  ( 39.58706461736021254, -291.0523547857346784, -270.3937649182068981 ) ) ;
#13319=CARTESIAN_POINT ( 'NONE',  ( 12.59191402391305914, -275.5735453205755903, -328.7631127921176812 ) ) ;
#13320=CARTESIAN_POINT ( 'NONE',  ( 34.71428584965417485, -293.2300723150740396, -258.5810196915511483 ) ) ;
#13321=CARTESIAN_POINT ( 'NONE',  ( 32.89800957462700381, -283.3670599640123555, -292.8229907658758293 ) ) ;
#13322=CARTESIAN_POINT ( 'NONE',  ( 20.66376293287339649, -277.7890978393866135, -316.0082958466583136 ) ) ;
#13323=CARTESIAN_POINT ( 'NONE',  ( -58.30751316631194925, -284.7430964692247244, -343.8943545077620456 ) ) ;
#13324=CARTESIAN_POINT ( 'NONE',  ( -48.40358893006416707, -281.9910141141397730, -342.9198191846614350 ) ) ;
#13325=CARTESIAN_POINT ( 'NONE',  ( -100.8556012367507719, -280.0150311124909877, -310.3452307262088539 ) ) ;
#13326=CARTESIAN_POINT ( 'NONE',  ( -113.5446204578502289, -272.8615831427289891, -258.9468195243208584 ) ) ;
#13327=CARTESIAN_POINT ( 'NONE',  ( 38.72794106646267664, -275.2351641450217130, -258.3425603676383275 ) ) ;
#13328=CARTESIAN_POINT ( 'NONE',  ( 35.74272605931487590, -295.6552476390149309, -284.5025765085347302 ) ) ;
#13332=CARTESIAN_POINT ( 'NONE',  ( -91.82548206730525919, -293.9587943249416071, -323.0092232242637920 ) ) ;
#13334=CARTESIAN_POINT ( 'NONE',  ( 35.76030458812795843, -275.0760287836251905, -271.5922547362052910 ) ) ;
#13335=CARTESIAN_POINT ( 'NONE',  ( -34.85764802893503145, -296.5415923271413590, -346.6273440562115411 ) ) ;
#13336=CARTESIAN_POINT ( 'NONE',  ( 38.42607710878368721, -294.8990354538168503, -281.6417496667460796 ) ) ;
#13337=CARTESIAN_POINT ( 'NONE',  ( -61.83153189358446156, -291.3713609529248743, -341.0737516871702155 ) ) ;
#13338=CARTESIAN_POINT ( 'NONE',  ( -71.30711949780425130, -275.5015684789742068, -337.0422901157353976 ) ) ;
#13339=CARTESIAN_POINT ( 'NONE',  ( -105.5818647435220470, -280.0786088314952167, -300.2323094017955327 ) ) ;
#13340=CARTESIAN_POINT ( 'NONE',  ( -108.2482811207109279, -294.3353342821780529, -293.1902690051132367 ) ) ;
#13341=CARTESIAN_POINT ( 'NONE',  ( 38.40471398893728860, -283.3709508381015212, -267.0867437688525570 ) ) ;
#13342=CARTESIAN_POINT ( 'NONE',  ( -109.4948291701508367, -283.6437434264569788, -257.3232252405673535 ) ) ;
#13343=CARTESIAN_POINT ( 'NONE',  ( 175.7829685710282490, 241.4225270720233993, -178.8902070973051650 ) ) ;
#13345=CARTESIAN_POINT ( 'NONE',  ( -101.0076760093505186, -284.7092620005935828, -234.4981560243688818 ) ) ;
#13347=CARTESIAN_POINT ( 'NONE',  ( 38.48696822839085740, -282.4835041891510059, -258.5495064154487750 ) ) ;
#13348=CARTESIAN_POINT ( 'NONE',  ( -112.7488796467082466, -283.1739298605095314, -284.1347429643098508 ) ) ;
#13349=CARTESIAN_POINT ( 'NONE',  ( -98.39652796683617453, -280.1158059992869767, -223.8087629838302632 ) ) ;
#13351=CARTESIAN_POINT ( 'NONE',  ( -73.74885610911908884, -279.0465600014897518, -337.4373486444525270 ) ) ;
#13352=CARTESIAN_POINT ( 'NONE',  ( -42.43160071744534889, -280.6409504488445350, -193.6316862197214732 ) ) ;
#13353=CARTESIAN_POINT ( 'NONE',  ( -107.3381139276884824, -270.1608578419545665, -262.4421837807431075 ) ) ;
#13354=CARTESIAN_POINT ( 'NONE',  ( 104.3268223557888632, 115.7811322214007106, -282.9140813606151710 ) ) ;
#13356=CARTESIAN_POINT ( 'NONE',  ( -4.526546245600342466, -276.4856637597059148, -203.0922537475019283 ) ) ;
#13357=CARTESIAN_POINT ( 'NONE',  ( 196.8892120694305561, 285.3822140004605217, -111.7264957686566760 ) ) ;
#13358=CARTESIAN_POINT ( 'NONE',  ( -24.57073831618998483, -278.2360412430826386, -196.8169181132106473 ) ) ;
#13359=CARTESIAN_POINT ( 'NONE',  ( 12.59545223515086043, -294.4973898731731197, -213.0876090509810581 ) ) ;
#13360=CARTESIAN_POINT ( 'NONE',  ( 31.90025972733708670, -292.5878521765746996, -246.7632736836748109 ) ) ;
#13361=CARTESIAN_POINT ( 'NONE',  ( -48.86597568641041534, -288.7026992182203458, -346.4855001391566702 ) ) ;
#13363=CARTESIAN_POINT ( 'NONE',  ( 34.92318372090718981, -292.4440451094114906, -295.3504073259857705 ) ) ;
#13364=CARTESIAN_POINT ( 'NONE',  ( -101.6788648948478624, -283.4426187345664516, -234.1016384298702633 ) ) ;
#13365=CARTESIAN_POINT ( 'NONE',  ( -49.92095674834108365, -293.7505379155027185, -197.1472666823371469 ) ) ;
#13366=CARTESIAN_POINT ( 'NONE',  ( -10.47937405178511838, -284.8889527304158378, -201.7244105465882740 ) ) ;
#13367=CARTESIAN_POINT ( 'NONE',  ( -10.78202387840521936, -284.0137163142777013, -338.9411714401007316 ) ) ;
#13369=CARTESIAN_POINT ( 'NONE',  ( -96.40553567100263876, -292.1549274917594516, -221.3073061160637849 ) ) ;
#13370=CARTESIAN_POINT ( 'NONE',  ( -24.04815227689346813, -283.3701023588765793, -342.2030975419046399 ) ) ;
#13371=CARTESIAN_POINT ( 'NONE',  ( 4.000022826579053614, -293.3038497304150951, -334.9128697508077721 ) ) ;
#13372=CARTESIAN_POINT ( 'NONE',  ( 33.89647625926698993, -288.7229474330244443, -299.3001277534231122 ) ) ;
#13373=CARTESIAN_POINT ( 'NONE',  ( -89.44519963789684880, -290.2554453254734881, -326.9716491752652132 ) ) ;
#13374=CARTESIAN_POINT ( 'NONE',  ( 20.33934892975745257, -287.0886295873547169, -225.6185590020763527 ) ) ;
#13376=CARTESIAN_POINT ( 'NONE',  ( -109.1670816552720140, -298.1039690335233558, -294.4737712642309475 ) ) ;
#13377=CARTESIAN_POINT ( 'NONE',  ( -35.46997145530772855, -296.7599569347117949, -193.8546733024735431 ) ) ;
#13378=CARTESIAN_POINT ( 'NONE',  ( -94.11536208669448911, -278.2636532426420217, -224.0992572687231075 ) ) ;
#13379=CARTESIAN_POINT ( 'NONE',  ( -104.1729650447399820, -272.5565160551118424, -232.1345486481228590 ) ) ;
#13380=CARTESIAN_POINT ( 'NONE',  ( -102.0855929066622423, -294.5561278674812797, -305.5596420800655437 ) ) ;
#13381=CARTESIAN_POINT ( 'NONE',  ( 36.11462389192714539, -277.4355523422403849, -279.8341022204190836 ) ) ;
#13382=CARTESIAN_POINT ( 'NONE',  ( -41.90878636754561626, -296.2336660129101915, -196.4888245454744151 ) ) ;
#13383=CARTESIAN_POINT ( 'NONE',  ( -69.88640781717172956, -296.6957617585835010, -336.1484458471023800 ) ) ;
#13384=CARTESIAN_POINT ( 'NONE',  ( -86.68794316496197894, -296.8374569706748503, -324.5752708490456371 ) ) ;
#13386=CARTESIAN_POINT ( 'NONE',  ( -39.06906525273071651, -296.6736123252691186, -346.5415395318700007 ) ) ;
#13387=CARTESIAN_POINT ( 'NONE',  ( -109.8467046344627818, -294.8085908945579945, -250.3434754030240299 ) ) ;
#13388=CARTESIAN_POINT ( 'NONE',  ( -1.213505996069036197, -293.1964363068412354, -206.7962790582370474 ) ) ;
#13389=CARTESIAN_POINT ( 'NONE',  ( -109.0196755427803907, -273.7080437808004945, -242.5301953407418978 ) ) ;
#13390=CARTESIAN_POINT ( 'NONE',  ( -89.08819371414298871, -288.3722507930980896, -322.6839172010979269 ) ) ;
#13391=CARTESIAN_POINT ( 'NONE',  ( -80.01335438358211150, -275.4753622634503358, -208.6203852425925618 ) ) ;
#13392=CARTESIAN_POINT ( 'NONE',  ( -38.36288823930932779, -274.5320166602838867, -193.4294334932374397 ) ) ;
#13393=CARTESIAN_POINT ( 'NONE',  ( -108.8007042618494182, -297.0843360651410308, -255.2777241437379416 ) ) ;
#13394=CARTESIAN_POINT ( 'NONE',  ( 31.65657358356577333, -283.1372703942421367, -240.0684616986798403 ) ) ;
#13395=CARTESIAN_POINT ( 'NONE',  ( -14.35983336860481430, -279.0287408646465224, -197.3320692362628392 ) ) ;
#13396=CARTESIAN_POINT ( 'NONE',  ( -27.39351775990539295, -282.2776311530182056, -346.6662700881418004 ) ) ;
#13397=CARTESIAN_POINT ( 'NONE',  ( 39.52113530922233764, -274.9469028837197015, -274.0473619053024095 ) ) ;
#13398=CARTESIAN_POINT ( 'NONE',  ( 25.63110975818091219, -279.3791782628262013, -227.3637065693968964 ) ) ;
#13399=CARTESIAN_POINT ( 'NONE',  ( -89.76095616019094336, -277.3149834530008206, -216.4160454584225306 ) ) ;
#13401=CARTESIAN_POINT ( 'NONE',  ( -40.78448521491121426, -272.5828642711813359, -196.8023618114719113 ) ) ;
#13402=CARTESIAN_POINT ( 'NONE',  ( 1.685545664834484203, -278.5308743098423179, -334.4663451851374703 ) ) ;
#13406=CARTESIAN_POINT ( 'NONE',  ( -99.08491283637989966, -295.3868079081368023, -226.0694743079803004 ) ) ;
#13407=CARTESIAN_POINT ( 'NONE',  ( -2.787112871733855801, -290.5266824355647373, -203.3810858706880822 ) ) ;
#13408=CARTESIAN_POINT ( 'NONE',  ( -77.16926297131196577, -291.5342045405558338, -204.3999652569031582 ) ) ;
#13409=CARTESIAN_POINT ( 'NONE',  ( 36.41477744666235594, -277.3666505435139129, -255.8693808431033858 ) ) ;
#13410=CARTESIAN_POINT ( 'NONE',  ( -49.16631192836808850, -271.9014379791024112, -196.2465487400072846 ) ) ;
#13412=CARTESIAN_POINT ( 'NONE',  ( 8.357681713831279779, -284.3522448830555618, -330.5348721822093694 ) ) ;
#13413=CARTESIAN_POINT ( 'NONE',  ( -112.1648252337331684, -282.6270792006542365, -264.5128473677176544 ) ) ;
#13415=CARTESIAN_POINT ( 'NONE',  ( 21.63643313585999195, -292.9563448865433202, -314.0499071902663673 ) ) ;
#13416=CARTESIAN_POINT ( 'NONE',  ( 19.62461394300983741, -285.0272024204127206, -222.7418884018648271 ) ) ;
#13418=CARTESIAN_POINT ( 'NONE',  ( -83.61320397315417097, -293.6862896726714780, -329.4523320296373754 ) ) ;
#13419=CARTESIAN_POINT ( 'NONE',  ( -113.6473458733575654, -283.0370184922652470, -269.9659240068711483 ) ) ;
#13420=CARTESIAN_POINT ( 'NONE',  ( -49.29129547746521212, -281.4974432588339255, -197.5349716856522377 ) ) ;
#13421=CARTESIAN_POINT ( 'NONE',  ( -113.8108999243323467, -285.6900414147070819, -275.7054469216830057 ) ) ;
#13422=CARTESIAN_POINT ( 'NONE',  ( 22.09687524660148128, -279.1495881088794704, -223.0009075289071063 ) ) ;
#13423=CARTESIAN_POINT ( 'NONE',  ( 28.22776145414211868, -287.9868029682542101, -302.4492109115161043 ) ) ;
#13424=CARTESIAN_POINT ( 'NONE',  ( -83.36121065967330424, -279.1220558802091887, -327.8512440487249933 ) ) ;
#13425=CARTESIAN_POINT ( 'NONE',  ( -91.42305940489916338, -280.0599531982767303, -221.0883231976278296 ) ) ;
#13426=CARTESIAN_POINT ( 'NONE',  ( -36.60734052983629994, -288.0412138422577186, -194.9967321662178108 ) ) ;
#13428=CARTESIAN_POINT ( 'NONE',  ( -95.56970503785156268, -297.0667602902819340, -219.8980202769687082 ) ) ;
#13429=CARTESIAN_POINT ( 'NONE',  ( 25.63937023511052260, -290.0737759971342484, -310.4264593361086781 ) ) ;
#13431=CARTESIAN_POINT ( 'NONE',  ( -37.37352853689063181, -276.5519495502701375, -190.3611179825600175 ) ) ;
#13433=CARTESIAN_POINT ( 'NONE',  ( -0.9111392813347855002, -272.5344510735800441, -204.5981512583235542 ) ) ;
#13435=CARTESIAN_POINT ( 'NONE',  ( 24.22772893737646882, -292.5544397841053410, -315.2790340227438719 ) ) ;
#13436=CARTESIAN_POINT ( 'NONE',  ( -109.6824026222367650, -272.0439004232600269, -259.4933110379953973 ) ) ;
#13437=CARTESIAN_POINT ( 'NONE',  ( 29.43007877499893254, -288.6551880316985148, -239.1803980963613583 ) ) ;
#13438=CARTESIAN_POINT ( 'NONE',  ( -2.694300823879401729, -282.2769208599086141, -204.9439034008434817 ) ) ;
#13439=CARTESIAN_POINT ( 'NONE',  ( -103.2807020242395453, -291.4698329008068640, -309.0747240418270394 ) ) ;
#13440=CARTESIAN_POINT ( 'NONE',  ( -82.54768766615792686, -290.9706569002191259, -332.0840226631880796 ) ) ;
#13441=CARTESIAN_POINT ( 'NONE',  ( -111.1660888676446319, -286.7230776760448521, -257.0614793527809070 ) ) ;
#13442=CARTESIAN_POINT ( 'NONE',  ( 6.182507220174499274, -280.7919689324610317, -206.8422752727321949 ) ) ;
#13443=CARTESIAN_POINT ( 'NONE',  ( 8.021756606764650854, -292.5172960263182631, -330.7885206101265680 ) ) ;
#13444=CARTESIAN_POINT ( 'NONE',  ( 10.82466232920867810, -280.5303210993626521, -210.2178094354298423 ) ) ;
#13445=CARTESIAN_POINT ( 'NONE',  ( 21.00780541608521901, -278.0493432586400218, -316.2749593928757577 ) ) ;
#13446=CARTESIAN_POINT ( 'NONE',  ( -95.95921662488163406, -298.4090924074130271, -317.1477375740089997 ) ) ;
#13447=CARTESIAN_POINT ( 'NONE',  ( 30.93479702270423815, -274.2273258260684088, -303.8319642929401425 ) ) ;
#13449=CARTESIAN_POINT ( 'NONE',  ( 30.38923339019997982, -281.4263598119951553, -297.7565388818734959 ) ) ;
#13450=CARTESIAN_POINT ( 'NONE',  ( -22.99812280010903365, -278.0777919906360012, -345.6630850139743529 ) ) ;
#13451=CARTESIAN_POINT ( 'NONE',  ( -46.25508524873569627, -275.2518853581394183, -197.4104836937257517 ) ) ;
#13452=CARTESIAN_POINT ( 'NONE',  ( -4.862571616127334018, -285.5282560630977855, -200.8059138270792232 ) ) ;
#13453=CARTESIAN_POINT ( 'NONE',  ( -90.56031213854326722, -293.0453471498078102, -218.9242309377517017 ) ) ;
#13454=CARTESIAN_POINT ( 'NONE',  ( -35.56310030641039788, -275.6742104319949362, -194.1688814032446544 ) ) ;
#13455=CARTESIAN_POINT ( 'NONE',  ( -35.55221805428152493, -275.3893021518002797, -193.8621512453394757 ) ) ;
#13457=CARTESIAN_POINT ( 'NONE',  ( -108.6075794412710422, -298.2550165231253914, -293.3585549387979654 ) ) ;
#13458=CARTESIAN_POINT ( 'NONE',  ( -37.57109341822355475, -281.0549083887496522, -345.2068460694425767 ) ) ;
#13459=CARTESIAN_POINT ( 'NONE',  ( -109.4525424624268766, -290.5613925118248630, -243.2691022053596726 ) ) ;
#13460=CARTESIAN_POINT ( 'NONE',  ( 20.28437203150357604, -272.9147228879465388, -222.9155427002361591 ) ) ;
#13461=CARTESIAN_POINT ( 'NONE',  ( -36.59396453843113761, -287.6615115858832041, -194.1518809281834024 ) ) ;
#13462=EDGE_CURVE ( 'NONE', #92893, #85445, #29349, .T. ) ;
#13463=CARTESIAN_POINT ( 'NONE',  ( -77.41266988040224817, -290.4208653339846933, -208.9726544388240086 ) ) ;
#13465=CARTESIAN_POINT ( 'NONE',  ( -109.3167036544355994, -288.7987872607223494, -296.1735964451011682 ) ) ;
#13466=CARTESIAN_POINT ( 'NONE',  ( -102.8662730884401242, -289.7823053697941305, -302.5887121378839311 ) ) ;
#13468=CARTESIAN_POINT ( 'NONE',  ( 21.26174044678009167, -289.3009245332277715, -319.8295853482165967 ) ) ;
#13469=CARTESIAN_POINT ( 'NONE',  ( -96.90048367997997047, -278.2954240465713838, -312.6301846521262178 ) ) ;
#13471=CARTESIAN_POINT ( 'NONE',  ( 8.709529664622065681, -293.3576434169266349, -331.6862901672117232 ) ) ;
#13472=CARTESIAN_POINT ( 'NONE',  ( -104.3241436687142283, -284.7115606680596898, -308.2401673304548240 ) ) ;
#13473=CARTESIAN_POINT ( 'NONE',  ( -114.1310962253205048, -284.9618296608421701, -264.2541438960388405 ) ) ;
#13474=CIRCLE ( 'NONE', #48235, 2.500000000000002220 ) ;
#13475=CARTESIAN_POINT ( 'NONE',  ( 32.98095433172179725, -282.1453069389218626, -290.0286484974020595 ) ) ;
#13476=CARTESIAN_POINT ( 'NONE',  ( 161.3244612304466159, 220.3882197354448351, -205.3170049622447380 ) ) ;
#13477=CARTESIAN_POINT ( 'NONE',  ( -114.3093106393634457, -272.1053998528684588, -270.3554297553863535 ) ) ;
#13478=CARTESIAN_POINT ( 'NONE',  ( 152.2530320059421172, 205.4471442928643796, -214.5373374589507875 ) ) ;
#13479=CARTESIAN_POINT ( 'NONE',  ( -94.73303068411735239, -272.3882235749208576, -224.9867099471016445 ) ) ;
#13480=CARTESIAN_POINT ( 'NONE',  ( -16.53984002476758874, -273.2475306711547205, -200.0123176032929564 ) ) ;
#13481=CARTESIAN_POINT ( 'NONE',  ( -69.50790991053510481, -294.9719039886864493, -340.2673269313805235 ) ) ;
#13482=CARTESIAN_POINT ( 'NONE',  ( -20.63144351428918810, -109.4982264660226576, -359.4589932074380840 ) ) ;
#13483=CARTESIAN_POINT ( 'NONE',  ( 2.177696442613713756, -273.2546344100842362, -204.8514578770309811 ) ) ;
#13484=CARTESIAN_POINT ( 'NONE',  ( -50.19060934628063109, -299.7468415103493271, -197.2463382883373697 ) ) ;
#13485=CARTESIAN_POINT ( 'NONE',  ( -65.45817679620414253, -292.7554010913407865, -202.6445925528496161 ) ) ;
#13486=ORIENTED_EDGE ( 'NONE', *, *, #75312, .F. ) ;
#13487=CARTESIAN_POINT ( 'NONE',  ( -109.2130038030962140, -297.1495119633174795, -297.4801917730546279 ) ) ;
#13488=CARTESIAN_POINT ( 'NONE',  ( 31.45945645978850180, -288.3715571168639826, -294.9454482309709533 ) ) ;
#13489=CARTESIAN_POINT ( 'NONE',  ( 4.148728207827702796, -295.3114345161935148, -335.0975886019558629 ) ) ;
#13490=CARTESIAN_POINT ( 'NONE',  ( -64.23879607682715687, -295.8862324646661364, -342.4449104238736368 ) ) ;
#13491=CARTESIAN_POINT ( 'NONE',  ( 35.64203388477530865, -293.7600669576484620, -273.4868538195490828 ) ) ;
#13493=CARTESIAN_POINT ( 'NONE',  ( 15.01136962998648627, -276.7038833034889080, -215.8774481058583490 ) ) ;
#13495=CARTESIAN_POINT ( 'NONE',  ( -112.9345415303678521, -278.2400050572518353, -255.9641669578193728 ) ) ;
#13496=CARTESIAN_POINT ( 'NONE',  ( 28.06607261930422581, -276.0477296939782264, -237.4182627388365177 ) ) ;
#13497=CARTESIAN_POINT ( 'NONE',  ( -35.57017976351612987, -275.8341973885931111, -194.3821433837524353 ) ) ;
#13498=CARTESIAN_POINT ( 'NONE',  ( 11.61645939648166781, -274.3966751625560505, -327.6455435786719477 ) ) ;
#13499=CARTESIAN_POINT ( 'NONE',  ( -72.90371501913402597, -298.2190285998299828, -206.4922228517793030 ) ) ;
#13500=CARTESIAN_POINT ( 'NONE',  ( -58.59562452442588665, -293.9071611937879993, -340.8142627927078934 ) ) ;
#13502=CARTESIAN_POINT ( 'NONE',  ( -101.8430560150894308, -279.5968424816661582, -228.3230530242886118 ) ) ;
#13503=CARTESIAN_POINT ( 'NONE',  ( 34.16499180440508354, -275.9126168619873738, -285.0510129244357813 ) ) ;
#13504=CARTESIAN_POINT ( 'NONE',  ( 19.92880294605765101, -285.5447086534340997, -219.5543232368817144 ) ) ;
#13505=CARTESIAN_POINT ( 'NONE',  ( 50.87328029350005210, -301.1541834273529616, -195.1644496284779677 ) ) ;
#13506=CARTESIAN_POINT ( 'NONE',  ( 82.67889722225095284, -297.1983528236896746, -196.2154390527394696 ) ) ;
#13507=CARTESIAN_POINT ( 'NONE',  ( 17.90482521173569097, -286.0670936331465555, -222.3983911501829880 ) ) ;
#13508=CARTESIAN_POINT ( 'NONE',  ( 18.74691343918777875, -279.1135153199455772, -222.0504407886007527 ) ) ;
#13509=CARTESIAN_POINT ( 'NONE',  ( -32.90953544718430379, -278.6838097926006981, -196.9054794376219490 ) ) ;
#13510=CARTESIAN_POINT ( 'NONE',  ( 37.53054988629661182, -289.6188008232904849, -275.5390759478623863 ) ) ;
#13511=CARTESIAN_POINT ( 'NONE',  ( 25.72455309725347661, -277.2706316976319840, -307.9081312897818066 ) ) ;
#13513=CARTESIAN_POINT ( 'NONE',  ( -12.22259462212732473, -274.9697639968247813, -342.1310461003222372 ) ) ;
#13514=CARTESIAN_POINT ( 'NONE',  ( 34.47208661321728584, -276.0235836508264242, -256.6982960807466156 ) ) ;
#13515=CARTESIAN_POINT ( 'NONE',  ( 22.27724916253489340, -282.9264981055762860, -224.5622743000091930 ) ) ;
#13516=EDGE_CURVE ( 'NONE', #17445, #16234, #6655, .T. ) ;
#13519=CARTESIAN_POINT ( 'NONE',  ( 20.40462421395662318, -290.1412712707963237, -319.0917677415128537 ) ) ;
#13520=CARTESIAN_POINT ( 'NONE',  ( 19.28000976063265171, -292.2350807588355224, -319.6207172758767570 ) ) ;
#13522=CARTESIAN_POINT ( 'NONE',  ( -0.2832286685470876697, -273.2408585354322668, -206.8805842461288478 ) ) ;
#13523=CARTESIAN_POINT ( 'NONE',  ( 27.32195216699895113, -291.1997340639658773, -233.7940983206480325 ) ) ;
#13524=CARTESIAN_POINT ( 'NONE',  ( 207.9738562182569979, 291.4636489450775798, -54.00000000000000711 ) ) ;
#13526=CARTESIAN_POINT ( 'NONE',  ( -86.94852856739331060, -288.2075733138581199, -328.4121739672628451 ) ) ;
#13527=CARTESIAN_POINT ( 'NONE',  ( 24.73045771854012997, -285.2040517441172938, -226.5092194211633512 ) ) ;
#13528=CARTESIAN_POINT ( 'NONE',  ( -94.73323218916556243, -285.3314873833873548, -316.4418447705828044 ) ) ;
#13529=CARTESIAN_POINT ( 'NONE',  ( -48.34289721544971030, -283.9985990840805243, -342.6907480745336443 ) ) ;
#13530=CARTESIAN_POINT ( 'NONE',  ( -83.28395150143130365, -293.4066108457627138, -210.5649731911737774 ) ) ;
#13532=CARTESIAN_POINT ( 'NONE',  ( -2.160298843411634806, -274.6699511095773119, -337.2310155755658911 ) ) ;
#13533=CARTESIAN_POINT ( 'NONE',  ( 2.403449765068615296, -274.9028237398029546, -204.4364082640365154 ) ) ;
#13534=CARTESIAN_POINT ( 'NONE',  ( -89.76885926844288122, -289.3996929548900425, -215.8761442644450881 ) ) ;
#13535=CARTESIAN_POINT ( 'NONE',  ( -97.05439269249619372, -277.8995837625887475, -318.9965197993265633 ) ) ;
#13536=CARTESIAN_POINT ( 'NONE',  ( -110.9815431279644145, -298.3745585545444214, -282.5685061910308491 ) ) ;
#13539=CARTESIAN_POINT ( 'NONE',  ( -91.87598027012479918, -283.9385504751987241, -221.0191736467336909 ) ) ;
#13540=CARTESIAN_POINT ( 'NONE',  ( -12.15633219618137417, -278.3795462078329024, -199.6617102941171140 ) ) ;
#13542=CARTESIAN_POINT ( 'NONE',  ( 17.60392472315898260, -273.2997933078729034, -217.3354019604138614 ) ) ;
#13543=CARTESIAN_POINT ( 'NONE',  ( -9.957867048168388635, -276.0334830791300647, -338.1538900878304617 ) ) ;
#13544=CARTESIAN_POINT ( 'NONE',  ( 27.77974248919749556, -295.5390377263745449, -304.9652207855666575 ) ) ;
#13545=CARTESIAN_POINT ( 'NONE',  ( 27.59696584744239445, -279.9350265949417462, -229.4637475159331359 ) ) ;
#13546=CARTESIAN_POINT ( 'NONE',  ( -9.129195875786994208, -295.6152360973462123, -337.9577774052037284 ) ) ;
#13547=CARTESIAN_POINT ( 'NONE',  ( -27.79267219791408650, -296.2486165386041534, -346.3226617902165003 ) ) ;
#13548=CARTESIAN_POINT ( 'NONE',  ( -40.51584640065840404, -297.8444832038135814, -197.4176100758153609 ) ) ;
#13549=CARTESIAN_POINT ( 'NONE',  ( -110.0535777945787856, -292.7890840132592984, -251.9244869546794519 ) ) ;
#13550=CARTESIAN_POINT ( 'NONE',  ( -114.3267303197576865, -284.7594099805384076, -267.1165243605342425 ) ) ;
#13551=CARTESIAN_POINT ( 'NONE',  ( -70.83508992561124273, -271.7546121252059947, -202.4015835200080744 ) ) ;
#13552=CARTESIAN_POINT ( 'NONE',  ( -36.56330013558817882, -285.8949894264509908, -193.3520135210320632 ) ) ;
#13553=CARTESIAN_POINT ( 'NONE',  ( -92.52950425866059447, -281.2368227782607164, -220.1002676227183485 ) ) ;
#13554=CARTESIAN_POINT ( 'NONE',  ( -65.17156383942467812, -284.7382118471848571, -202.5656685514693436 ) ) ;
#13555=CARTESIAN_POINT ( 'NONE',  ( -99.04992516383904899, -287.9740693113418502, -312.9885224604685163 ) ) ;
#13556=CARTESIAN_POINT ( 'NONE',  ( 181.0595704366054690, 252.2700355933461651, -164.3583243123303532 ) ) ;
#13557=CARTESIAN_POINT ( 'NONE',  ( -14.54085261312238408, -285.8633414116842459, -200.8954475590673212 ) ) ;
#13558=CARTESIAN_POINT ( 'NONE',  ( -18.96307513166993530, -283.7625496074473972, -344.9480931306172806 ) ) ;
#13559=CARTESIAN_POINT ( 'NONE',  ( -99.83251601703139499, -290.2032452199792374, -225.7772852312661485 ) ) ;
#13560=CARTESIAN_POINT ( 'NONE',  ( -67.06934635342329898, -281.2690270038789322, -200.1991092711630529 ) ) ;
#13561=CARTESIAN_POINT ( 'NONE',  ( -111.6919312326862581, -279.6395943707336755, -288.4531644820152678 ) ) ;
#13562=CARTESIAN_POINT ( 'NONE',  ( 7.144005322061190100, -280.5105622456058541, -212.4177844322115334 ) ) ;
#13563=CARTESIAN_POINT ( 'NONE',  ( 35.77807340377263046, -277.3373698500812452, -253.6154860658987218 ) ) ;
#13564=CARTESIAN_POINT ( 'NONE',  ( -93.68946994483439994, -295.8366181018540715, -322.8584262593573726 ) ) ;
#13565=CARTESIAN_POINT ( 'NONE',  ( -71.95741865491031319, -287.5321977798403168, -336.5087509784855229 ) ) ;
#13566=CARTESIAN_POINT ( 'NONE',  ( -95.52605175127334292, -296.0974704478106219, -225.7446226865440622 ) ) ;
#13569=CARTESIAN_POINT ( 'NONE',  ( -34.77282814818167367, -284.9398170641782713, -344.7694654354556860 ) ) ;
#13570=CARTESIAN_POINT ( 'NONE',  ( -108.9062948670838864, -296.0266673669443662, -284.9353404755230486 ) ) ;
#13571=CARTESIAN_POINT ( 'NONE',  ( 36.78026919083271196, -294.3838242233839537, -250.6273429870099392 ) ) ;
#13572=CARTESIAN_POINT ( 'NONE',  ( -82.85170864116497569, -284.3447430437678918, -327.6338618906827378 ) ) ;
#13573=CARTESIAN_POINT ( 'NONE',  ( -0.1489144665720578964, -273.5931885471683813, -203.1932328212933783 ) ) ;
#13574=CARTESIAN_POINT ( 'NONE',  ( 7.881276161537572378, -289.1040618707446583, -332.6216034741153749 ) ) ;
#13575=CARTESIAN_POINT ( 'NONE',  ( -96.22759931379648890, -282.0417459461705789, -318.0549475543778044 ) ) ;
#13576=CARTESIAN_POINT ( 'NONE',  ( -107.7103179318719555, -290.4855756983972128, -301.7012089019423797 ) ) ;
#13577=CARTESIAN_POINT ( 'NONE',  ( -13.27690408578824410, -289.0640583405504458, -339.3029273451480208 ) ) ;
#13580=CARTESIAN_POINT ( 'NONE',  ( 64.89032082630019715, 46.31952104162717632, -315.2875490666531277 ) ) ;
#13581=CARTESIAN_POINT ( 'NONE',  ( -110.4683760289727132, -287.8380690714490129, -287.0191576251351080 ) ) ;
#13583=CARTESIAN_POINT ( 'NONE',  ( 11.52204353826855332, -279.6695816220120037, -215.7116840629992396 ) ) ;
#13584=CARTESIAN_POINT ( 'NONE',  ( 21.83732480571998025, -274.5565534830449792, -221.1311748634412879 ) ) ;
#13585=CARTESIAN_POINT ( 'NONE',  ( -48.86564649644491709, -279.1992999849621810, -344.3544948652295261 ) ) ;
#13586=CARTESIAN_POINT ( 'NONE',  ( -10.91761978339317452, -93.10046803755994915, -357.6389493721724762 ) ) ;
#13587=CARTESIAN_POINT ( 'NONE',  ( 29.23949249098504666, -280.6182974651587756, -307.9595883749491350 ) ) ;
#13588=CARTESIAN_POINT ( 'NONE',  ( 4.287065625126643020, -280.5083902097566124, -332.3824254439375636 ) ) ;
#13589=CARTESIAN_POINT ( 'NONE',  ( -109.8529884865901636, -298.6035312422611128, -247.4689788413477913 ) ) ;
#13590=CARTESIAN_POINT ( 'NONE',  ( 17.13063089981426401, -294.7405982199778123, -319.0703672003883185 ) ) ;
#13592=CARTESIAN_POINT ( 'NONE',  ( -109.1481313034094853, -289.0311349668756975, -286.0747124883238826 ) ) ;
#13593=CARTESIAN_POINT ( 'NONE',  ( -41.19597260903686475, -274.6563820257134125, -193.5075125659404875 ) ) ;
#13594=CARTESIAN_POINT ( 'NONE',  ( -104.3797064758031325, -272.9419661265707191, -241.3382807244666139 ) ) ;
#13599=CARTESIAN_POINT ( 'NONE',  ( 19.06517424551938333, -281.9703343784356662, -223.5176013457259785 ) ) ;
#13600=CARTESIAN_POINT ( 'NONE',  ( -2.870138647403114085, -282.2615066253839586, -202.6288964700407575 ) ) ;
#13602=CARTESIAN_POINT ( 'NONE',  ( -108.2534988450514106, -283.8517119234795132, -252.0601548530923992 ) ) ;
#13603=CARTESIAN_POINT ( 'NONE',  ( -21.96123867709017574, -282.1115884320992109, -197.6839628719043276 ) ) ;
#13604=CARTESIAN_POINT ( 'NONE',  ( 33.90762946340650075, -274.2782208065635245, -289.1824034511878381 ) ) ;
#13607=CARTESIAN_POINT ( 'NONE',  ( -59.60842893775332385, -278.1362424746458828, -343.9026138077355768 ) ) ;
#13611=CARTESIAN_POINT ( 'NONE',  ( -34.51487717437815661, -284.9966714366802876, -345.6632818113504868 ) ) ;
#13612=CARTESIAN_POINT ( 'NONE',  ( 34.64389043881742936, -292.5764393517611666, -257.2270819024182060 ) ) ;
#13613=CARTESIAN_POINT ( 'NONE',  ( -51.67444999180394660, -288.5794835329385251, -345.9116644241893823 ) ) ;
#13614=CARTESIAN_POINT ( 'NONE',  ( -107.4855755694752446, -283.1033375590394030, -246.5827677832739369 ) ) ;
#13615=CARTESIAN_POINT ( 'NONE',  ( -91.94634617264296139, -283.8284699686502677, -220.9536436097992578 ) ) ;
#13616=CARTESIAN_POINT ( 'NONE',  ( -59.00686868212586234, -287.5760540205180860, -341.1860850154860145 ) ) ;
#13617=CARTESIAN_POINT ( 'NONE',  ( -5.848719225844257963, -283.8337708325140056, -336.6721738225040781 ) ) ;
#13618=CARTESIAN_POINT ( 'NONE',  ( 30.74831331479195740, -273.1375551194737454, -238.7929471153562417 ) ) ;
#13619=CARTESIAN_POINT ( 'NONE',  ( -112.2083134290982258, -283.1348102441622245, -255.8943486732702581 ) ) ;
#13620=CARTESIAN_POINT ( 'NONE',  ( -89.30747421619737736, -297.7833327776335750, -324.5117861945354321 ) ) ;
#13621=CARTESIAN_POINT ( 'NONE',  ( 0.6183570199544879964, -284.5567248697578293, -205.4688542527828474 ) ) ;
#13622=CARTESIAN_POINT ( 'NONE',  ( -109.7227936589355721, -279.3467563468761909, -281.5139538366073566 ) ) ;
#13623=CARTESIAN_POINT ( 'NONE',  ( 10.88142246406368230, -288.7170840258521594, -212.6342301019168701 ) ) ;
#13628=CARTESIAN_POINT ( 'NONE',  ( 23.73696742204157673, -296.0741533896636497, -314.8656212193303077 ) ) ;
#13629=CARTESIAN_POINT ( 'NONE',  ( -111.8949662158130280, -276.4411255330553558, -278.9954447842501963 ) ) ;
#13630=CARTESIAN_POINT ( 'NONE',  ( -99.06875761925890345, -290.3591839925926479, -224.5796092927287191 ) ) ;
#13631=CARTESIAN_POINT ( 'NONE',  ( 26.47433489965567333, -292.4550618215052395, -307.4280046479551061 ) ) ;
#13632=CARTESIAN_POINT ( 'NONE',  ( -7.785853932361445295, -279.1325913649729955, -203.0591992792633675 ) ) ;
#13633=CARTESIAN_POINT ( 'NONE',  ( -77.31733040410809110, -271.5913096368487913, -207.5657106607734761 ) ) ;
#13634=CARTESIAN_POINT ( 'NONE',  ( -101.5627074419343217, -292.3538836556028286, -234.5227331140128513 ) ) ;
#13635=CARTESIAN_POINT ( 'NONE',  ( -85.33152481854862970, -281.9090924074130839, -210.2361428286348826 ) ) ;
#13636=CARTESIAN_POINT ( 'NONE',  ( -19.46863260694070519, -293.3063195641213383, -344.5994749119380458 ) ) ;
#13637=CARTESIAN_POINT ( 'NONE',  ( 22.62349163323107604, -289.7471043955331993, -313.3799068230014768 ) ) ;
#13638=CARTESIAN_POINT ( 'NONE',  ( 1.205639248390016460, -290.7989103079572146, -204.8175700132173063 ) ) ;
#13639=CARTESIAN_POINT ( 'NONE',  ( -107.5693236899448380, -292.2669988261392859, -248.3310058580287034 ) ) ;
#13641=CARTESIAN_POINT ( 'NONE',  ( -36.21387402543916068, -292.8694486054196773, -197.1958302686302886 ) ) ;
#13643=CARTESIAN_POINT ( 'NONE',  ( -113.2746579064918961, -291.8891979233982852, -259.8630643500327437 ) ) ;
#13644=CARTESIAN_POINT ( 'NONE',  ( 20.33448348700062880, -280.2395526681830233, -318.8571451360037941 ) ) ;
#13645=CARTESIAN_POINT ( 'NONE',  ( 18.47658724361285820, -292.8837535087899937, -223.3151957906105451 ) ) ;
#13646=CARTESIAN_POINT ( 'NONE',  ( 1.373973389439363757, -280.5540929698765353, -203.7414417187063975 ) ) ;
#13647=CARTESIAN_POINT ( 'NONE',  ( 19.76497235415774156, -281.9207065076909657, -322.0585938682344818 ) ) ;
#13648=CARTESIAN_POINT ( 'NONE',  ( -1.200860039792204459, -284.5310798962817671, -204.5849545870420059 ) ) ;
#13649=CARTESIAN_POINT ( 'NONE',  ( 33.15698741160961305, -279.3862654943009147, -246.9438226472128122 ) ) ;
#13650=CARTESIAN_POINT ( 'NONE',  ( -103.6516099054150288, -283.0178173562750317, -235.2072095585744762 ) ) ;
#13652=CARTESIAN_POINT ( 'NONE',  ( 14.70273203987860100, -279.2487375289848615, -214.4848832783396517 ) ) ;
#13653=CARTESIAN_POINT ( 'NONE',  ( -73.45524823339481202, -284.5052301921081721, -202.6465284059426324 ) ) ;
#13654=CARTESIAN_POINT ( 'NONE',  ( -1.652774354567535298, -275.3408660899337974, -206.4804892536207603 ) ) ;
#13656=CARTESIAN_POINT ( 'NONE',  ( -12.00448043137212295, -293.9874806121997608, -200.9924027580908614 ) ) ;
#13657=CARTESIAN_POINT ( 'NONE',  ( -15.95977647059763882, -275.7485460722206199, -196.9480469432443215 ) ) ;
#13658=CARTESIAN_POINT ( 'NONE',  ( -61.80090498741567728, -277.0455669578506672, -339.2177444549793108 ) ) ;
#13659=CARTESIAN_POINT ( 'NONE',  ( -111.9215034743445898, -290.4785412741468349, -289.5672643941420574 ) ) ;
#13660=CARTESIAN_POINT ( 'NONE',  ( 35.79177982547468417, -279.8742767763482675, -289.3560728585725315 ) ) ;
#13661=CARTESIAN_POINT ( 'NONE',  ( -13.86443462074993249, -292.1817741386894909, -196.9715348642621393 ) ) ;
#13662=CIRCLE ( 'NONE', #80220, 6.154241149514405151 ) ;
#13663=CARTESIAN_POINT ( 'NONE',  ( -99.90641824617176781, -290.1334969489502669, -232.2945382229105462 ) ) ;
#13664=CARTESIAN_POINT ( 'NONE',  ( 3.126151351717162186, -292.5088930849533426, -333.5677475182520766 ) ) ;
#13667=CARTESIAN_POINT ( 'NONE',  ( -3.602269449905252774, -292.0177838136859236, -205.5564942329011728 ) ) ;
#13670=CARTESIAN_POINT ( 'NONE',  ( -37.37352853689063181, -280.5523547857346784, -340.3611179825599606 ) ) ;
#13671=CARTESIAN_POINT ( 'NONE',  ( -89.43979183231243724, -296.3986071571849834, -213.9099674330401513 ) ) ;
#13672=CARTESIAN_POINT ( 'NONE',  ( -109.7524993311614878, -285.5541248229128541, -295.0587784193310767 ) ) ;
#13673=CARTESIAN_POINT ( 'NONE',  ( 16.89203854658096660, -286.6856223635634819, -221.4783421779349055 ) ) ;
#13674=CARTESIAN_POINT ( 'NONE',  ( 36.29577892867075661, -277.1241564719789494, -274.3308617939764531 ) ) ;
#13675=CARTESIAN_POINT ( 'NONE',  ( -89.67255134133135641, -293.8142032484376500, -323.6628049503987654 ) ) ;
#13676=CARTESIAN_POINT ( 'NONE',  ( -68.92973617321707991, -297.2333787808157695, -337.3091103341832877 ) ) ;
#13677=CARTESIAN_POINT ( 'NONE',  ( 1.066202684958064362, -275.3223662342861076, -332.9665215625577162 ) ) ;
#13680=CARTESIAN_POINT ( 'NONE',  ( -114.3451773695185523, -296.1925527361041759, -272.4649786494220507 ) ) ;
#13681=CARTESIAN_POINT ( 'NONE',  ( -10.17624887484230811, -290.6150761644905742, -339.7226338035293338 ) ) ;
#13682=CARTESIAN_POINT ( 'NONE',  ( -38.45329906659297592, -296.0380649664108432, -195.3662034614006870 ) ) ;
#13684=CARTESIAN_POINT ( 'NONE',  ( 17.06483578370574605, -279.8632155322168273, -216.1317071792590809 ) ) ;
#13685=CARTESIAN_POINT ( 'NONE',  ( -58.81489195178848206, -295.9740993578237749, -344.2557291067359415 ) ) ;
#13686=CARTESIAN_POINT ( 'NONE',  ( -95.45906256776146392, -288.0267678487963963, -318.9886320374207571 ) ) ;
#13687=CARTESIAN_POINT ( 'NONE',  ( -111.5705032566660577, -296.6299238462630115, -290.7530055282207400 ) ) ;
#13688=CARTESIAN_POINT ( 'NONE',  ( -0.08381094472334088552, -292.8960675533546123, -207.5603442582150819 ) ) ;
#13692=CARTESIAN_POINT ( 'NONE',  ( -67.75955034644672992, -290.9642795826238739, -340.3429880788557966 ) ) ;
#13693=CARTESIAN_POINT ( 'NONE',  ( 35.65787339142939771, -296.4086741954485547, -190.3901485728259217 ) ) ;
#13695=CARTESIAN_POINT ( 'NONE',  ( -8.891102911485702975, -279.7632998165365166, -198.9196992910592030 ) ) ;
#13696=CARTESIAN_POINT ( 'NONE',  ( -101.9720056611995744, -286.0472506389759815, -308.0831543949820457 ) ) ;
#13697=CARTESIAN_POINT ( 'NONE',  ( -29.50518370236875754, -284.7242987085503501, -194.3532545561998859 ) ) ;
#13698=CARTESIAN_POINT ( 'NONE',  ( -7.666487825732072992, -286.7401244687881672, -338.6855036344348946 ) ) ;
#13699=CARTESIAN_POINT ( 'NONE',  ( 31.42188628798750472, -276.9975103334746223, -238.4262893452703622 ) ) ;
#13701=CARTESIAN_POINT ( 'NONE',  ( -83.00675806506637855, -277.6970129023891900, -327.3796877340411697 ) ) ;
#13702=CARTESIAN_POINT ( 'NONE',  ( -107.3223024918708006, -278.1801442563533442, -249.2280169064609368 ) ) ;
#13703=CARTESIAN_POINT ( 'NONE',  ( 15.80289339776934021, -275.8635360488769379, -215.0696657665166924 ) ) ;
#13704=CARTESIAN_POINT ( 'NONE',  ( -67.19349695917806287, -278.4642760872553140, -199.8141198524807294 ) ) ;
#13705=CARTESIAN_POINT ( 'NONE',  ( -78.63461375671516862, -207.3269539590848751, -354.3927223517632683 ) ) ;
#13706=CARTESIAN_POINT ( 'NONE',  ( -38.36632987209058854, -274.9808488121906862, -193.6032496701160142 ) ) ;
#13707=CARTESIAN_POINT ( 'NONE',  ( -80.30880217689754375, -298.9081948954108157, -207.1117779230685301 ) ) ;
#13708=CARTESIAN_POINT ( 'NONE',  ( -37.30987171927208124, -291.5519495502701943, -345.3611179825600175 ) ) ;
#13710=DIRECTION ( 'NONE',  ( 0.000000000000000000, 1.000000000000000000, -1.224646799147353207E-16 ) ) ;
#13711=CARTESIAN_POINT ( 'NONE',  ( 9.216257597466716689, -287.7890620028209696, -213.7344224665082777 ) ) ;
#13712=CARTESIAN_POINT ( 'NONE',  ( -82.68934215043969971, -287.2024122755286726, -209.3236482214858540 ) ) ;
#13713=CARTESIAN_POINT ( 'NONE',  ( -34.58245312017958639, -288.3652924627605785, -343.4606100419794075 ) ) ;
#13714=CARTESIAN_POINT ( 'NONE',  ( -110.1684554879753932, -283.7468950378806198, -295.1762465721661783 ) ) ;
#13715=CARTESIAN_POINT ( 'NONE',  ( -35.62397099359790786, -278.4738950980721484, -196.5685699317976116 ) ) ;
#13716=CARTESIAN_POINT ( 'NONE',  ( -24.95871440880734582, -288.0720333736266525, -197.1138233734441769 ) ) ;
#13717=CARTESIAN_POINT ( 'NONE',  ( 35.82578007256254438, -280.1522813798314360, -279.5638461576048712 ) ) ;
#13718=CARTESIAN_POINT ( 'NONE',  ( 7.897045284182422797, -277.7347459944202228, -328.3457433943577257 ) ) ;
#13719=CARTESIAN_POINT ( 'NONE',  ( 35.70430180562726719, -276.0246438604691548, -268.8544518083155594 ) ) ;
#13720=CARTESIAN_POINT ( 'NONE',  ( 31.32464673198284544, -286.7870503003185263, -304.4356923307113902 ) ) ;
#13722=CARTESIAN_POINT ( 'NONE',  ( -63.84670351252362508, -284.1919843359269748, -342.4835390174972645 ) ) ;
#13723=CARTESIAN_POINT ( 'NONE',  ( -63.88489860875980497, -283.8815490215756085, -342.5759746091673037 ) ) ;
#13724=CARTESIAN_POINT ( 'NONE',  ( -34.31545332652866875, -280.2579005600961750, -197.4113285917850646 ) ) ;
#13728=CARTESIAN_POINT ( 'NONE',  ( -4.841090942817596776, -290.4891506201363995, -338.8152383476980276 ) ) ;
#13730=CARTESIAN_POINT ( 'NONE',  ( -99.47959105461899298, -288.6413400722894380, -315.0174222178917489 ) ) ;
#13731=CARTESIAN_POINT ( 'NONE',  ( -104.5910301538779521, -272.0008656080828473, -241.2337538751546617 ) ) ;
#13733=CARTESIAN_POINT ( 'NONE',  ( 37.96378059450398013, -292.7049623297373273, -254.7274315520643313 ) ) ;
#13735=CARTESIAN_POINT ( 'NONE',  ( -109.3442708911288008, -288.8262202221503117, -286.1149974315113127 ) ) ;
#13736=CARTESIAN_POINT ( 'NONE',  ( 20.14686314483438423, -291.1413440135990527, -223.7251976090080063 ) ) ;
#13737=CARTESIAN_POINT ( 'NONE',  ( 34.09105620740524500, -288.9785406157570833, -287.2280035422941182 ) ) ;
#13738=CARTESIAN_POINT ( 'NONE',  ( -4.829096099716510437, -288.9805209788416391, -202.7746430608542312 ) ) ;
#13739=CARTESIAN_POINT ( 'NONE',  ( -37.47186702827235649, -291.0539023648515240, -345.3737421144371069 ) ) ;
#13740=CARTESIAN_POINT ( 'NONE',  ( -111.3621068081675816, -288.7195278116091117, -257.2841220243305997 ) ) ;
#13742=CARTESIAN_POINT ( 'NONE',  ( -37.26740574209865287, -294.0532745998751807, -195.3485791444505537 ) ) ;
#13743=CARTESIAN_POINT ( 'NONE',  ( -109.7290635677364179, -285.3430187533374465, -281.7981982519130497 ) ) ;
#13744=CARTESIAN_POINT ( 'NONE',  ( -25.33987449247666746, -294.2049700456593087, -196.1587958794362123 ) ) ;
#13745=CARTESIAN_POINT ( 'NONE',  ( -114.3366298191176895, -272.7563261381201301, -270.3637176062232470 ) ) ;
#13746=EDGE_CURVE ( 'NONE', #36646, #41846, #72444, .T. ) ;
#13748=CARTESIAN_POINT ( 'NONE',  ( -9.790537445922979032, -300.3146391628407628, -194.7921782358073415 ) ) ;
#13749=CARTESIAN_POINT ( 'NONE',  ( -5.972965751319449623, -281.8261878425273608, -336.4703156422215216 ) ) ;
#13750=CARTESIAN_POINT ( 'NONE',  ( -1.494546149260095325, -280.5767895270439567, -336.2543377224904475 ) ) ;
#13751=CARTESIAN_POINT ( 'NONE',  ( -109.2899514968314776, -295.4057083103001560, -297.4854969212216247 ) ) ;
#13752=CARTESIAN_POINT ( 'NONE',  ( -43.54501353716532464, -272.2127128057708774, -196.5567857530153617 ) ) ;
#13753=CARTESIAN_POINT ( 'NONE',  ( -111.3382062549010101, -276.5211190551790992, -278.9317982136229261 ) ) ;
#13754=CARTESIAN_POINT ( 'NONE',  ( -110.2275319208518169, -297.9959224510134277, -260.5473801730598780 ) ) ;
#13755=CARTESIAN_POINT ( 'NONE',  ( 15.63170791097852685, -273.3589959267579843, -215.2936654122469804 ) ) ;
#13756=CARTESIAN_POINT ( 'NONE',  ( -75.95188054528840382, -297.0036902640176208, -333.0673772392078718 ) ) ;
#13758=CARTESIAN_POINT ( 'NONE',  ( -106.1355369150969921, -297.0222443726284496, -295.4100190807086506 ) ) ;
#13760=CARTESIAN_POINT ( 'NONE',  ( 34.80321528886052818, -285.8518676814848618, -292.1663517381721249 ) ) ;
#13761=CARTESIAN_POINT ( 'NONE',  ( -78.85332748939212877, -273.3088706031089714, -210.2515292568515690 ) ) ;
#13762=CARTESIAN_POINT ( 'NONE',  ( -69.79283926952251704, -285.6365930307589451, -200.5189388990921771 ) ) ;
#13763=CARTESIAN_POINT ( 'NONE',  ( 34.02113396979854087, -287.5870165811727475, -299.3663821283937523 ) ) ;
#13764=CARTESIAN_POINT ( 'NONE',  ( -92.47689600519227326, -299.2481988400395494, -218.9184804145422731 ) ) ;
#13765=CARTESIAN_POINT ( 'NONE',  ( -22.34903732883500993, -290.2444268882245524, -197.0450318511009584 ) ) ;
#13766=CARTESIAN_POINT ( 'NONE',  ( -64.67530590450131456, -278.9014880006275234, -198.4925261815276656 ) ) ;
#13767=CARTESIAN_POINT ( 'NONE',  ( -106.6662871844225293, -287.6237833571633473, -303.7098442033569654 ) ) ;
#13768=CARTESIAN_POINT ( 'NONE',  ( 34.38730498677439584, -286.1429363136008419, -254.8021870629456487 ) ) ;
#13770=CARTESIAN_POINT ( 'NONE',  ( -40.05533752652011259, -287.0859725880587803, -345.3629529728368084 ) ) ;
#13771=CARTESIAN_POINT ( 'NONE',  ( -44.66856687509758217, -299.5581668526814951, -196.8747872970527624 ) ) ;
#13772=CARTESIAN_POINT ( 'NONE',  ( -7.781824385329735527, -281.8572617504339632, -199.8854468587001350 ) ) ;
#13773=CARTESIAN_POINT ( 'NONE',  ( -96.91773870222317555, -295.2019843947819027, -224.1981049282061065 ) ) ;
#13774=CARTESIAN_POINT ( 'NONE',  ( 35.56592173907153409, -281.6005831265100028, -274.0324493046078373 ) ) ;
#13775=CARTESIAN_POINT ( 'NONE',  ( -110.3450346168987579, -296.4105062578059346, -294.8460757733156470 ) ) ;
#13776=CARTESIAN_POINT ( 'NONE',  ( -109.1135704158158291, -274.1901189571070745, -254.1077012780311293 ) ) ;
#13777=CARTESIAN_POINT ( 'NONE',  ( -14.85239196843773612, -282.3435414664533596, -198.7578698140214044 ) ) ;
#13778=CARTESIAN_POINT ( 'NONE',  ( -101.4146484076270269, -296.0941204872580101, -234.8918954609972616 ) ) ;
#13780=FACE_OUTER_BOUND ( 'NONE', #65492, .T. ) ;
#13781=CARTESIAN_POINT ( 'NONE',  ( 23.15956195591534694, -284.1303887461084514, -314.1030776364909229 ) ) ;
#13783=CARTESIAN_POINT ( 'NONE',  ( -95.95921662488163406, -294.6952119285919025, -223.5744983911110353 ) ) ;
#13784=CARTESIAN_POINT ( 'NONE',  ( 38.33486201150012107, -274.5815416878353403, -256.9736004814580497 ) ) ;
#13785=CARTESIAN_POINT ( 'NONE',  ( 22.58914744273794639, -292.8042727447717084, -228.6582391455953029 ) ) ;
#13786=CARTESIAN_POINT ( 'NONE',  ( 15.74553495893989741, -282.3404799172340063, -219.1760779527031957 ) ) ;
#13787=CARTESIAN_POINT ( 'NONE',  ( 36.40241823385852626, -277.2041500127876361, -274.3356198848738359 ) ) ;
#13788=CARTESIAN_POINT ( 'NONE',  ( -108.7458018565789502, -285.6287319254290082, -297.7125166024455325 ) ) ;
#13789=CARTESIAN_POINT ( 'NONE',  ( 29.33981347029352449, -279.9340937798414188, -239.5683264877759200 ) ) ;
#13790=CARTESIAN_POINT ( 'NONE',  ( -111.2528157938226485, -280.3878400213831696, -283.1706004541239281 ) ) ;
#13791=CARTESIAN_POINT ( 'NONE',  ( -34.04695977709405952, -298.0923358081694232, -193.3611179127478863 ) ) ;
#13792=CARTESIAN_POINT ( 'NONE',  ( 21.72926089983860010, -276.0501701793031089, -319.7536434066195739 ) ) ;
#13793=CARTESIAN_POINT ( 'NONE',  ( 31.93448154075495538, -295.8312016574400900, -297.7442376404128481 ) ) ;
#13796=CARTESIAN_POINT ( 'NONE',  ( -99.72003015995909436, -295.2690186796248781, -227.3354281492931648 ) ) ;
#13797=CARTESIAN_POINT ( 'NONE',  ( 13.54400666820939314, -274.2961896977533911, -217.9337083058065616 ) ) ;
#13799=CARTESIAN_POINT ( 'NONE',  ( 38.74823860038389967, -294.9997442242173520, -264.6140338863293096 ) ) ;
#13800=CARTESIAN_POINT ( 'NONE',  ( 39.31426275336387732, -294.7563941697390533, -270.2949048963678251 ) ) ;
#13801=CARTESIAN_POINT ( 'NONE',  ( 2.303917721861872714, -290.5198157394684131, -333.8296409751218903 ) ) ;
#13802=CARTESIAN_POINT ( 'NONE',  ( -84.17343999460125303, -275.6971742504012468, -328.7957690127227579 ) ) ;
#13803=CARTESIAN_POINT ( 'NONE',  ( 17.61036962121105631, -278.1788373003473112, -320.5955155483267163 ) ) ;
#13804=CARTESIAN_POINT ( 'NONE',  ( -104.0696179844612885, -294.1920264653994082, -303.4731203355949560 ) ) ;
#13805=CARTESIAN_POINT ( 'NONE',  ( 36.77136814797378150, -283.2117914317101395, -254.5651467127682395 ) ) ;
#13806=CARTESIAN_POINT ( 'NONE',  ( -39.97129539926085329, -284.9386632195789275, -197.0991817329320099 ) ) ;
#13807=CARTESIAN_POINT ( 'NONE',  ( 86.53115587608755277, 81.67541019969276306, -301.2104785531669791 ) ) ;
#13809=CARTESIAN_POINT ( 'NONE',  ( -79.31797053866654323, -285.1350133261153132, -210.5488968255646967 ) ) ;
#13810=CARTESIAN_POINT ( 'NONE',  ( -6.367867214589843172, -281.5292141867943201, -200.1891237866793460 ) ) ;
#13811=CARTESIAN_POINT ( 'NONE',  ( -104.0786642346094908, -282.8553706178260541, -308.0742596360763628 ) ) ;
#13812=CARTESIAN_POINT ( 'NONE',  ( -113.4853041314929101, -279.6207330724033113, -260.2108971320544697 ) ) ;
#13814=CARTESIAN_POINT ( 'NONE',  ( -62.16200719779108397, -278.8891471615843898, -342.5741041693481748 ) ) ;
#13815=CARTESIAN_POINT ( 'NONE',  ( 26.47324843497312585, -301.4082689599840705, -200.3320873922942553 ) ) ;
#13816=CARTESIAN_POINT ( 'NONE',  ( 169.2043900173948714, 231.8925807357131248, -192.6779440976073090 ) ) ;
#13818=CARTESIAN_POINT ( 'NONE',  ( -109.7196847477654273, -274.7995226233286417, -251.1501716192047127 ) ) ;
#13819=CARTESIAN_POINT ( 'NONE',  ( -84.45682939641071130, -277.4204115232868730, -212.3976785749237877 ) ) ;
#13820=CARTESIAN_POINT ( 'NONE',  ( -87.99094461473853812, -293.1151726275268175, -213.7163649639146570 ) ) ;
#13821=CARTESIAN_POINT ( 'NONE',  ( 34.93748526230803719, -293.0491426060059439, -281.6268590439194099 ) ) ;
#13822=CARTESIAN_POINT ( 'NONE',  ( -112.2042710200168045, -289.8369153488018242, -288.1691947544702543 ) ) ;
#13824=CARTESIAN_POINT ( 'NONE',  ( 6.262751130153954016, -293.0479373284229609, -333.1731531567143634 ) ) ;
#13825=CARTESIAN_POINT ( 'NONE',  ( 9.554378471220637437, -285.1096934725891856, -213.3769252179830573 ) ) ;
#13826=CARTESIAN_POINT ( 'NONE',  ( -19.80292938901446576, -294.1402999932092257, -198.1743629054663529 ) ) ;
#13827=CARTESIAN_POINT ( 'NONE',  ( -7.960900414601150388, -284.9241031374633621, -202.7780109070870083 ) ) ;
#13828=CARTESIAN_POINT ( 'NONE',  ( 3.679272258087318281, -283.8029257854306593, -331.4023813106707621 ) ) ;
#13830=CARTESIAN_POINT ( 'NONE',  ( -13.94959483957682878, -293.2895277274598129, -197.1915042597769911 ) ) ;
#13831=CARTESIAN_POINT ( 'NONE',  ( 27.83345613268470231, -281.5952272979674831, -237.2309714127197822 ) ) ;
#13832=CARTESIAN_POINT ( 'NONE',  ( 39.10475045691349294, -292.4182820575210258, -276.0251519761974350 ) ) ;
#13833=CARTESIAN_POINT ( 'NONE',  ( -67.98007853865773598, -290.2471061334842375, -340.8270571961376163 ) ) ;
#13834=CARTESIAN_POINT ( 'NONE',  ( -114.1895314914742556, -290.9977705905373000, -274.0944432849754548 ) ) ;
#13835=CARTESIAN_POINT ( 'NONE',  ( 24.94961695304684923, -287.1944060393321365, -232.2981199294274006 ) ) ;
#13836=ORIENTED_EDGE ( 'NONE', *, *, #56608, .T. ) ;
#13838=CARTESIAN_POINT ( 'NONE',  ( 23.90202860175057609, -296.0144249183804277, -314.9869170896032529 ) ) ;
#13839=CARTESIAN_POINT ( 'NONE',  ( -99.51098442883292705, -295.8317032346340056, -225.7710029013032909 ) ) ;
#13840=CARTESIAN_POINT ( 'NONE',  ( -104.4919118862638356, -277.2176632504560985, -299.7159230139587294 ) ) ;
#13842=CARTESIAN_POINT ( 'NONE',  ( -105.5514804762074164, -272.5206439725981795, -234.6517084826563462 ) ) ;
#13843=CARTESIAN_POINT ( 'NONE',  ( -68.83101988011340211, -293.9536470956139169, -337.0017811404400163 ) ) ;
#13844=CARTESIAN_POINT ( 'NONE',  ( 29.99884081982527562, -276.9024110634111935, -239.5252425068507023 ) ) ;
#13845=CARTESIAN_POINT ( 'NONE',  ( -51.77887032122603728, -272.0052037540064021, -197.4906445287676320 ) ) ;
#13846=CARTESIAN_POINT ( 'NONE',  ( 17.38683348229893966, -295.4532116487959001, -319.2873114987274334 ) ) ;
#13847=CARTESIAN_POINT ( 'NONE',  ( -53.20291669239951204, -296.3398828731852177, -341.9859963003457892 ) ) ;
#13849=CARTESIAN_POINT ( 'NONE',  ( -110.8185687409976055, -294.3489524106902309, -286.2097207507188728 ) ) ;
#13850=CARTESIAN_POINT ( 'NONE',  ( -112.2880544601896702, -273.5673719416994913, -253.4140594250813763 ) ) ;
#13851=CARTESIAN_POINT ( 'NONE',  ( 23.22462044429903116, -286.7046300548752811, -312.1815962561309448 ) ) ;
#13852=CARTESIAN_POINT ( 'NONE',  ( -35.36239268324980145, -276.0771255025746882, -195.3743876976912475 ) ) ;
#13853=CARTESIAN_POINT ( 'NONE',  ( -97.76863161707223071, -273.6819678508643392, -222.7364095383559857 ) ) ;
#13854=CARTESIAN_POINT ( 'NONE',  ( -106.8881074978329480, -296.5884060691602144, -292.7820167008665067 ) ) ;
#13855=CARTESIAN_POINT ( 'NONE',  ( -91.90067697950352965, -281.2588173906169686, -218.3084166985720458 ) ) ;
#13856=CARTESIAN_POINT ( 'NONE',  ( -22.64440197356533346, -278.9211762468011671, -195.2253347856420760 ) ) ;
#13857=CARTESIAN_POINT ( 'NONE',  ( -18.95082437226056271, -282.1701406969540926, -345.0825166320857988 ) ) ;
#13858=CARTESIAN_POINT ( 'NONE',  ( 39.45306623616082931, -274.8392956770359206, -265.4545597158873420 ) ) ;
#13859=CARTESIAN_POINT ( 'NONE',  ( 35.83720117554236850, -279.6823015463204456, -249.0707367076533671 ) ) ;
#13860=CARTESIAN_POINT ( 'NONE',  ( -35.35825355495023103, -278.0768060958984620, -195.2077966996185694 ) ) ;
#13862=CARTESIAN_POINT ( 'NONE',  ( 5.534673921256747953, -273.2199133480867772, -210.4901708934459066 ) ) ;
#13863=CARTESIAN_POINT ( 'NONE',  ( 35.69911773042250047, -277.3329289820165400, -253.2753318245520404 ) ) ;
#13865=CARTESIAN_POINT ( 'NONE',  ( -55.76179165756899181, -289.8364141939027832, -197.2381553244462395 ) ) ;
#13867=CARTESIAN_POINT ( 'NONE',  ( -97.46356613883708064, -291.1965560023747344, -222.2533095998791737 ) ) ;
#13869=CARTESIAN_POINT ( 'NONE',  ( -28.78385074413047917, -278.9441809993283528, -345.0913384605607916 ) ) ;
#13870=CARTESIAN_POINT ( 'NONE',  ( -35.31133640963481923, -272.0774514690457977, -195.3757535277878503 ) ) ;
#13873=CARTESIAN_POINT ( 'NONE',  ( -63.12829348636812909, -283.7162859271044795, -199.8789987046618535 ) ) ;
#13875=CARTESIAN_POINT ( 'NONE',  ( -9.092159207519776132, -293.4692550630706478, -338.1176480249738461 ) ) ;
#13876=CARTESIAN_POINT ( 'NONE',  ( 34.89770183830172812, -285.9135452394748427, -287.4589040187652813 ) ) ;
#13879=CARTESIAN_POINT ( 'NONE',  ( -69.39460006631520628, -293.4736863239355102, -338.1809221109065220 ) ) ;
#13880=CARTESIAN_POINT ( 'NONE',  ( -112.9155006348995727, -282.8941703488339385, -281.2852848898040747 ) ) ;
#13881=CARTESIAN_POINT ( 'NONE',  ( -108.3940014747174985, -280.4136804977609927, -250.3640227833301992 ) ) ;
#13882=CARTESIAN_POINT ( 'NONE',  ( -97.27935688356468802, -286.3991526854563858, -222.6590632746684832 ) ) ;
#13883=CARTESIAN_POINT ( 'NONE',  ( 37.26409516417955103, -279.6092633698817167, -255.9406698379628153 ) ) ;
#13884=CARTESIAN_POINT ( 'NONE',  ( 32.66996914282456999, -287.2780763744044066, -249.6441852604225744 ) ) ;
#13885=CARTESIAN_POINT ( 'NONE',  ( -76.65538895197525449, -279.0144663504079290, -332.6288273084067555 ) ) ;
#13886=CARTESIAN_POINT ( 'NONE',  ( -94.57297022161840516, -278.7125370842812231, -315.9572539577405337 ) ) ;
#13887=CARTESIAN_POINT ( 'NONE',  ( -35.22035727339236644, -288.0585190858773785, -195.0229159501386107 ) ) ;
#13889=CARTESIAN_POINT ( 'NONE',  ( -35.46978037339534495, -297.9083036264289035, -193.3611691524987179 ) ) ;
#13890=CARTESIAN_POINT ( 'NONE',  ( -10.10086472495352083, -290.6748046522712912, -339.9132089729552604 ) ) ;
#13891=CARTESIAN_POINT ( 'NONE',  ( 133.0872704186301405, -299.5541904835127980, -202.0153591320744226 ) ) ;
#13892=CARTESIAN_POINT ( 'NONE',  ( -19.05039376806008633, -285.3376638359844719, -350.3538533559490702 ) ) ;
#13894=CARTESIAN_POINT ( 'NONE',  ( 28.35779963562260875, -273.0658602049711590, -233.7354773566951565 ) ) ;
#13895=CARTESIAN_POINT ( 'NONE',  ( 20.71430914698659720, -291.2794607579100443, -220.9859322173466580 ) ) ;
#13896=CARTESIAN_POINT ( 'NONE',  ( -102.8260960304365597, -295.6196035908107547, -302.8758095803309516 ) ) ;
#13897=CARTESIAN_POINT ( 'NONE',  ( -37.29973151637383211, -287.5727738013668500, -196.6552370485001973 ) ) ;
#13898=CARTESIAN_POINT ( 'NONE',  ( 22.13002728783479967, -282.7027397504519399, -226.2820191376268326 ) ) ;
#13899=CARTESIAN_POINT ( 'NONE',  ( -29.02314814989797043, -290.3740885136897418, -346.3708543099326107 ) ) ;
#13900=CARTESIAN_POINT ( 'NONE',  ( -84.84528372748631853, -291.0064737556717773, -330.4012583873403628 ) ) ;
#13901=CARTESIAN_POINT ( 'NONE',  ( -100.7075165172649207, -286.0114868524486837, -310.5802809824875226 ) ) ;
#13902=CARTESIAN_POINT ( 'NONE',  ( -51.31053502479835515, -277.3927069767499916, -346.0834505939782844 ) ) ;
#13904=CARTESIAN_POINT ( 'NONE',  ( -61.16125358079393237, -293.4387307106679827, -342.1231647293279252 ) ) ;
#13905=CARTESIAN_POINT ( 'NONE',  ( 39.18302242493180643, -281.2728021034162680, -261.3520736238132827 ) ) ;
#13906=CARTESIAN_POINT ( 'NONE',  ( -109.7447831794055588, -274.6251921393022712, -253.9702958932091974 ) ) ;
#13907=CARTESIAN_POINT ( 'NONE',  ( -85.28047601435908120, -292.1948066931273615, -330.5268031993605859 ) ) ;
#13908=CARTESIAN_POINT ( 'NONE',  ( 28.21030407220004577, -274.2989388077428998, -308.7916885913560350 ) ) ;
#13910=CARTESIAN_POINT ( 'NONE',  ( 11.35149465784171774, -280.2568112751799276, -215.8912986048921994 ) ) ;
#13911=CARTESIAN_POINT ( 'NONE',  ( -17.44616398114765587, -278.0060325726952328, -344.3352780585476012 ) ) ;
#13912=CARTESIAN_POINT ( 'NONE',  ( -104.2619236311069102, -298.3884015333197794, -239.6269870349098312 ) ) ;
#13913=CARTESIAN_POINT ( 'NONE',  ( -63.84206929732978608, -282.4481810269372772, -342.4065942226606580 ) ) ;
#13914=CARTESIAN_POINT ( 'NONE',  ( -91.31659424574539230, -291.5927785683759339, -321.0786537339303663 ) ) ;
#13915=CARTESIAN_POINT ( 'NONE',  ( -65.94601730740606627, -275.2842163509899933, -199.7196661012601453 ) ) ;
#13916=CARTESIAN_POINT ( 'NONE',  ( -111.3456117824015053, -274.1141762646116717, -250.7489374756198686 ) ) ;
#13918=CARTESIAN_POINT ( 'NONE',  ( 31.17870385544242851, -295.9470949751941475, -300.4440477184514293 ) ) ;
#13919=CARTESIAN_POINT ( 'NONE',  ( -32.04062742820021725, -280.9849457042334393, -345.0064598027554439 ) ) ;
#13920=CARTESIAN_POINT ( 'NONE',  ( -112.2431038817852880, -289.9959555951043626, -288.1805269029781016 ) ) ;
#13921=CARTESIAN_POINT ( 'NONE',  ( 34.08306152892657082, -273.8536245856207074, -292.0929357077902750 ) ) ;
#13922=CARTESIAN_POINT ( 'NONE',  ( 30.69822059083624310, -288.7061592649998829, -236.0535444457762821 ) ) ;
#13923=CARTESIAN_POINT ( 'NONE',  ( -108.4047378986518595, -289.7097502756898848, -252.3025838715099383 ) ) ;
#13925=CARTESIAN_POINT ( 'NONE',  ( -99.40238966083316541, -288.5312595766996537, -314.9601852023115498 ) ) ;
#13926=CARTESIAN_POINT ( 'NONE',  ( -72.63344644033401210, -291.2382316069362105, -206.3779344886439731 ) ) ;
#13928=CARTESIAN_POINT ( 'NONE',  ( 22.17399736623949735, -289.2835070508272111, -318.7488687464811505 ) ) ;
#13929=CARTESIAN_POINT ( 'NONE',  ( 19.20066113503581917, -276.5396825521901860, -316.5874120009416970 ) ) ;
#13931=CARTESIAN_POINT ( 'NONE',  ( -71.94690938237734201, -294.4192572883148387, -338.8006679767718197 ) ) ;
#13932=CARTESIAN_POINT ( 'NONE',  ( -102.8269252101145383, -284.6759829311966996, -310.6723829387304932 ) ) ;
#13933=CARTESIAN_POINT ( 'NONE',  ( -107.9084469141536715, -285.2791603305217905, -239.4694301635275338 ) ) ;
#13934=CARTESIAN_POINT ( 'NONE',  ( 34.50701660207009525, -282.0582311665448856, -283.4638320346683713 ) ) ;
#13935=CARTESIAN_POINT ( 'NONE',  ( 45.02227103420001697, 12.57429608517253961, -332.0372542094538062 ) ) ;
#13937=CARTESIAN_POINT ( 'NONE',  ( 192.8964254566477905, 279.1718055284784441, -125.5694871102472376 ) ) ;
#13938=CARTESIAN_POINT ( 'NONE',  ( -22.61259601301798483, -108.4505377025144242, -359.0006681345822130 ) ) ;
#13939=( GEOMETRIC_REPRESENTATION_CONTEXT ( 3 ) GLOBAL_UNCERTAINTY_ASSIGNED_CONTEXT ( ( #39591 ) ) GLOBAL_UNIT_ASSIGNED_CONTEXT ( ( #78729, #64089, #43208 ) ) REPRESENTATION_CONTEXT ( 'NONE', 'WORKASPACE' ) );
#13940=CARTESIAN_POINT ( 'NONE',  ( -92.13232101574408262, -272.4405000909766272, -221.8782386332586043 ) ) ;
#13941=CARTESIAN_POINT ( 'NONE',  ( -48.91071740801071854, -272.8217788585934613, -197.9192328261104876 ) ) ;
#13942=CARTESIAN_POINT ( 'NONE',  ( -70.78679458155451698, -294.9891162679484751, -339.6645234084620597 ) ) ;
#13943=CARTESIAN_POINT ( 'NONE',  ( -87.79732207361467999, -230.1314203361037301, -344.7605846467396304 ) ) ;
#13944=CARTESIAN_POINT ( 'NONE',  ( -31.28231389223850556, -272.8119750995933259, -194.0814013717944988 ) ) ;
#13945=CARTESIAN_POINT ( 'NONE',  ( -109.6860279954746602, -298.6285320421354186, -253.7128835571040781 ) ) ;
#13946=CARTESIAN_POINT ( 'NONE',  ( 12.50248238604651796, -289.6556378521762554, -324.4377017862967705 ) ) ;
#13947=CARTESIAN_POINT ( 'NONE',  ( -102.6913282385188637, -292.0824498205961959, -237.0274441948036781 ) ) ;
#13949=CARTESIAN_POINT ( 'NONE',  ( -102.9083715996914492, -296.9704828890004364, -310.2839410876592297 ) ) ;
#13951=CARTESIAN_POINT ( 'NONE',  ( 15.06927833456615851, -287.3091378701336680, -219.4584876160160150 ) ) ;
#13952=CARTESIAN_POINT ( 'NONE',  ( 29.43940176766727745, -294.8507760003695921, -308.4744588754392680 ) ) ;
#13953=CARTESIAN_POINT ( 'NONE',  ( -34.85035099077237675, -295.5139837230917692, -347.2592329327564471 ) ) ;
#13954=CARTESIAN_POINT ( 'NONE',  ( -1.258522564495346163, -292.7117813842300507, -206.8879610891251843 ) ) ;
#13956=CARTESIAN_POINT ( 'NONE',  ( -16.20408140379166895, -276.2433481790006908, -197.7636239889024523 ) ) ;
#13959=CARTESIAN_POINT ( 'NONE',  ( -114.3234301369553805, -278.0442852626783292, -271.6011420763450133 ) ) ;
#13960=CARTESIAN_POINT ( 'NONE',  ( 34.94408123618173789, -274.1460942670458962, -285.2341213691066741 ) ) ;
#13961=CARTESIAN_POINT ( 'NONE',  ( 24.18856565479102017, -277.0425723235796909, -310.1715809883531847 ) ) ;
#13962=CARTESIAN_POINT ( 'NONE',  ( -49.57844098909943398, -275.6584560164728259, -195.3131111677384126 ) ) ;
#13963=CARTESIAN_POINT ( 'NONE',  ( 27.66404565220688738, -274.0792232336564211, -308.4748926090412056 ) ) ;
#13964=CARTESIAN_POINT ( 'NONE',  ( -44.58743185363938011, -298.6096046369905253, -197.5687104263188587 ) ) ;
#13965=CARTESIAN_POINT ( 'NONE',  ( -38.36857645374530534, -293.6399992249069442, -343.9431840307071298 ) ) ;
#13967=CARTESIAN_POINT ( 'NONE',  ( -98.75051561006894474, -278.4264690647755174, -316.7344837930183417 ) ) ;
#13968=CARTESIAN_POINT ( 'NONE',  ( 17.43663486931767181, -276.4080388961909307, -318.6327903016679102 ) ) ;
#13969=CARTESIAN_POINT ( 'NONE',  ( -40.77745235512595912, -284.6947503035688101, -193.8795922955957565 ) ) ;
#13970=CARTESIAN_POINT ( 'NONE',  ( -56.93693582120787511, -299.8003121437577647, -197.7395603548327756 ) ) ;
#13971=CARTESIAN_POINT ( 'NONE',  ( 82.63805641362395704, -300.4059824324262422, -197.7175201709814019 ) ) ;
#13972=CARTESIAN_POINT ( 'NONE',  ( 23.63845033345183566, -287.3092787066311189, -310.8070461044287072 ) ) ;
#13974=CARTESIAN_POINT ( 'NONE',  ( -72.59287493551462944, -277.8185007445991346, -205.2817150226913725 ) ) ;
#13975=CARTESIAN_POINT ( 'NONE',  ( -49.21928027160467423, -278.4725296819978553, -197.7367556394873986 ) ) ;
#13976=CARTESIAN_POINT ( 'NONE',  ( -110.5803792769081042, -286.3441510188929442, -286.5777818089525226 ) ) ;
#13977=CARTESIAN_POINT ( 'NONE',  ( -21.55272684444882714, -278.0504086211623758, -342.0921152256848359 ) ) ;
#13979=CARTESIAN_POINT ( 'NONE',  ( 36.86060554855468041, -273.7323197756792865, -252.9705596984334477 ) ) ;
#13980=CARTESIAN_POINT ( 'NONE',  ( 32.95574599036767438, -275.9366329000378641, -250.1263459734549599 ) ) ;
#13981=CARTESIAN_POINT ( 'NONE',  ( 36.86219651193465552, -283.7069798689504978, -282.4337731464697754 ) ) ;
#13983=CARTESIAN_POINT ( 'NONE',  ( 19.50596705572998601, -290.1586888761673890, -320.1566857630890013 ) ) ;
#13984=CARTESIAN_POINT ( 'NONE',  ( 28.68944520935930242, -292.0253808842684862, -306.0345839285895408 ) ) ;
#13986=CARTESIAN_POINT ( 'NONE',  ( -40.78136994951938732, -272.6929447662913049, -196.8984651037467870 ) ) ;
#13987=CARTESIAN_POINT ( 'NONE',  ( 35.53248676140506745, -291.8752888915151971, -284.5109719674903204 ) ) ;
#13988=CARTESIAN_POINT ( 'NONE',  ( 121.1498776811041438, 150.0802918209077177, -263.8330885344481658 ) ) ;
#13990=CARTESIAN_POINT ( 'NONE',  ( -43.14901327210228033, -287.6041061774054697, -346.4464836372922036 ) ) ;
#13991=CARTESIAN_POINT ( 'NONE',  ( -5.182169578036499580, -284.7094993623931600, -201.5153584037910264 ) ) ;
#13992=CARTESIAN_POINT ( 'NONE',  ( -18.56793586405532182, -284.2309807281924350, -341.5681525110846906 ) ) ;
#13994=CARTESIAN_POINT ( 'NONE',  ( -101.9089367386394258, -284.8858792272508254, -304.8734732437175694 ) ) ;
#13995=CARTESIAN_POINT ( 'NONE',  ( -76.34009215513137292, -293.5137774700590398, -205.8220001725522366 ) ) ;
#13996=CARTESIAN_POINT ( 'NONE',  ( 35.21022174696152263, -273.3601485704849665, -249.0704178336520442 ) ) ;
#13998=CARTESIAN_POINT ( 'NONE',  ( 21.83188142953161659, -275.2230080161028241, -221.1246321486615614 ) ) ;
#14000=CARTESIAN_POINT ( 'NONE',  ( -103.8993110872538495, -288.1607531927754167, -306.1298000775723267 ) ) ;
#14001=CARTESIAN_POINT ( 'NONE',  ( -70.30101726200295786, -277.4745387684100706, -339.9649469544103795 ) ) ;
#14002=CARTESIAN_POINT ( 'NONE',  ( 35.94392880358793008, -295.7149761097521150, -284.5408005424354769 ) ) ;
#14005=CARTESIAN_POINT ( 'NONE',  ( -110.8840263982265242, -283.2299583353841399, -270.8962879372326711 ) ) ;
#14006=CARTESIAN_POINT ( 'NONE',  ( -96.97035648470519220, -277.1748693203211928, -224.8492839413438560 ) ) ;
#14007=CARTESIAN_POINT ( 'NONE',  ( 52.43474621377098543, -297.5582050755576233, -194.1850537549212561 ) ) ;
#14008=CARTESIAN_POINT ( 'NONE',  ( -41.87117731851381564, -276.4592829566884689, -343.3352047031388565 ) ) ;
#14010=CARTESIAN_POINT ( 'NONE',  ( -19.92691529862905853, -293.8000607818966046, -198.7022591221019070 ) ) ;
#14011=CARTESIAN_POINT ( 'NONE',  ( 18.64875676080346523, -293.8248532635283254, -223.1543686121119379 ) ) ;
#14012=CARTESIAN_POINT ( 'NONE',  ( -55.93412788960144866, -296.6019039335914158, -344.5744584367828907 ) ) ;
#14013=CARTESIAN_POINT ( 'NONE',  ( -97.18459369217598010, -295.8025314269007708, -312.1681520126081182 ) ) ;
#14014=CARTESIAN_POINT ( 'NONE',  ( -4.905012468922741675, -290.6251904419686980, -337.9840574882693431 ) ) ;
#14015=CARTESIAN_POINT ( 'NONE',  ( -107.0047416322343992, -284.2986503617667040, -303.1644814210063714 ) ) ;
#14016=CARTESIAN_POINT ( 'NONE',  ( -16.10057293618129748, -272.4633867731518535, -197.5803246476255026 ) ) ;
#14017=CARTESIAN_POINT ( 'NONE',  ( 31.42274725833685878, -286.9396351998213959, -235.7135959914429861 ) ) ;
#14018=CARTESIAN_POINT ( 'NONE',  ( -110.0835700105092627, -280.3152574682040381, -287.1648363960576376 ) ) ;
#14019=CARTESIAN_POINT ( 'NONE',  ( -79.43475759041217543, -284.5271403797784728, -210.3690505390151486 ) ) ;
#14020=CARTESIAN_POINT ( 'NONE',  ( -86.10395804379319884, -287.7276120369754722, -327.4139369828311033 ) ) ;
#14021=CARTESIAN_POINT ( 'NONE',  ( 201.7648208617462728, 289.3015991269851384, -82.29596988341933184 ) ) ;
#14022=CARTESIAN_POINT ( 'NONE',  ( -19.79501048500039673, -285.7915498532761376, -199.4379051109754641 ) ) ;
#14023=CARTESIAN_POINT ( 'NONE',  ( -21.76199643385749027, -283.7984002363313607, -345.5282187985935707 ) ) ;
#14024=CARTESIAN_POINT ( 'NONE',  ( -95.47486193030424317, -290.2901610347151404, -220.2076508610878989 ) ) ;
#14025=CARTESIAN_POINT ( 'NONE',  ( -72.15963582219853834, -281.1995835920613445, -202.5664448791465588 ) ) ;
#14026=CARTESIAN_POINT ( 'NONE',  ( -113.8912042552325374, -279.8515156087285050, -271.6171234615896424 ) ) ;
#14027=CARTESIAN_POINT ( 'NONE',  ( 30.33373449885391793, -281.7519745318558080, -297.7296318724862658 ) ) ;
#14028=CARTESIAN_POINT ( 'NONE',  ( -63.91532113618128363, -275.6838174916088633, -200.5928241190977985 ) ) ;
#14029=CARTESIAN_POINT ( 'NONE',  ( -3.228783570963782878, -294.6141346856778682, -339.4069389610562553 ) ) ;
#14030=CARTESIAN_POINT ( 'NONE',  ( -51.07834888656000061, -287.2485352606307174, -343.7839262310250774 ) ) ;
#14031=CARTESIAN_POINT ( 'NONE',  ( -86.01782091859632828, -292.9909627607779612, -211.6660119433807949 ) ) ;
#14032=CARTESIAN_POINT ( 'NONE',  ( -95.85934710826388994, -294.8545690630814988, -314.5395992957853650 ) ) ;
#14034=CARTESIAN_POINT ( 'NONE',  ( 16.89142717854064557, -284.1928122744155871, -321.4265136511351102 ) ) ;
#14035=CARTESIAN_POINT ( 'NONE',  ( -92.20936670838629823, -295.5312630572193484, -318.5443790890765285 ) ) ;
#14036=CARTESIAN_POINT ( 'NONE',  ( -3.470313686029046885, -293.5684616275291319, -201.5409595524095892 ) ) ;
#14037=CARTESIAN_POINT ( 'NONE',  ( -3.108692801777531045, -281.1683720528533286, -205.7559474921650065 ) ) ;
#14038=CARTESIAN_POINT ( 'NONE',  ( -67.43233360154476941, -272.7257408847764850, -199.7397756663388009 ) ) ;
#14039=CARTESIAN_POINT ( 'NONE',  ( -85.09487544735820563, -290.3428197588968942, -330.7029841899748703 ) ) ;
#14040=CARTESIAN_POINT ( 'NONE',  ( 1.441180044896873902, -280.6792731409850035, -335.4471663006981998 ) ) ;
#14041=CARTESIAN_POINT ( 'NONE',  ( -100.0163013263131973, -291.4775725279130256, -225.6661668560507792 ) ) ;
#14042=CARTESIAN_POINT ( 'NONE',  ( -0.9772292964629729628, -288.8887809096349315, -333.7416143040517795 ) ) ;
#14045=CARTESIAN_POINT ( 'NONE',  ( 45.42119675738224061, 10.99673322031138412, -328.3769721457455830 ) ) ;
#14046=CARTESIAN_POINT ( 'NONE',  ( 90.38368222445549804, -297.2649936051623740, -200.4191791630918829 ) ) ;
#14047=CARTESIAN_POINT ( 'NONE',  ( -108.6459449522204466, -277.5329834346950975, -286.7967320428482481 ) ) ;
#14049=CARTESIAN_POINT ( 'NONE',  ( -24.81008966536818861, -279.1361170996223677, -198.1310355237392002 ) ) ;
#14050=CARTESIAN_POINT ( 'NONE',  ( 39.60208087879163941, -275.2649837109509008, -274.0471857123279165 ) ) ;
#14051=CARTESIAN_POINT ( 'NONE',  ( 204.1739257889963426, 292.3637011233957992, -68.35704339179807221 ) ) ;
#14052=CARTESIAN_POINT ( 'NONE',  ( -48.01835787157568802, -278.4937470192833757, -194.6464996853970604 ) ) ;
#14053=CARTESIAN_POINT ( 'NONE',  ( -6.598580490294386536, -280.6666100292207489, -338.3950424086135058 ) ) ;
#14054=CARTESIAN_POINT ( 'NONE',  ( -113.2978551945238195, -298.3573562008087379, -266.8053500766753814 ) ) ;
#14055=CARTESIAN_POINT ( 'NONE',  ( 22.63486968089157259, -293.4631935817392900, -228.6161875331386568 ) ) ;
#14057=CARTESIAN_POINT ( 'NONE',  ( -58.84933899805359658, -288.0209495837702889, -340.6899185866644757 ) ) ;
#14058=CARTESIAN_POINT ( 'NONE',  ( 38.62561297402739058, -276.0531253393550060, -258.3481752850842668 ) ) ;
#14059=CARTESIAN_POINT ( 'NONE',  ( -34.48206726786463605, -298.2556126639216245, -197.3610342856659372 ) ) ;
#14066=CARTESIAN_POINT ( 'NONE',  ( -74.67499940345929588, -280.6227553722633843, -207.2119506859932017 ) ) ;
#14067=CARTESIAN_POINT ( 'NONE',  ( -7.949922215315155860, -282.1920765836794089, -200.2749179418074732 ) ) ;
#14068=CARTESIAN_POINT ( 'NONE',  ( -104.3333517805514816, -283.2139805525881115, -299.9504244342596735 ) ) ;
#14069=CARTESIAN_POINT ( 'NONE',  ( -52.09564324425033277, -281.7218604765699865, -197.5542197944056966 ) ) ;
#14070=CARTESIAN_POINT ( 'NONE',  ( 19.70614025917264556, -274.6865793893451269, -317.0313084605385257 ) ) ;
#14075=CARTESIAN_POINT ( 'NONE',  ( -11.90996338542509037, -277.5323247366557666, -342.9247617639934447 ) ) ;
#14077=CARTESIAN_POINT ( 'NONE',  ( -28.68594959952024226, -275.5193002513117335, -346.3332146333099217 ) ) ;
#14080=CARTESIAN_POINT ( 'NONE',  ( -109.9007486375338374, -286.2716373934872536, -290.6980618046380869 ) ) ;
#14082=CARTESIAN_POINT ( 'NONE',  ( 21.45014514778553405, -293.3585230118524692, -313.9055855579143213 ) ) ;
#14083=CARTESIAN_POINT ( 'NONE',  ( 39.24518048515181334, -286.9872872705570899, -277.2721601839047594 ) ) ;
#14084=CARTESIAN_POINT ( 'NONE',  ( -111.0005955772205510, -282.8926971637777115, -262.6221195037292659 ) ) ;
#14085=CARTESIAN_POINT ( 'NONE',  ( -54.87931107184501656, -284.3971077231576032, -198.8394768870798828 ) ) ;
#14086=CARTESIAN_POINT ( 'NONE',  ( -70.44555980785480642, -287.7345165263075160, -336.5726681701117968 ) ) ;
#14087=CARTESIAN_POINT ( 'NONE',  ( -7.075795367499152277, -283.8510627892477487, -337.2412334445056672 ) ) ;
#14088=CARTESIAN_POINT ( 'NONE',  ( -34.16181914077959192, -272.0919910481815123, -195.4285549145483856 ) ) ;
#14089=CARTESIAN_POINT ( 'NONE',  ( -113.4111493182427779, -282.8852889598923639, -275.6418252806089981 ) ) ;
#14090=CARTESIAN_POINT ( 'NONE',  ( -68.66870370198434159, -297.4640084013508954, -338.5192818797780774 ) ) ;
#14091=CARTESIAN_POINT ( 'NONE',  ( -8.033873317821269566, -284.4348554751310871, -201.0881757254733770 ) ) ;
#14093=CARTESIAN_POINT ( 'NONE',  ( -107.8480839875027613, -279.7549105419758462, -250.5090994207240271 ) ) ;
#14094=CARTESIAN_POINT ( 'NONE',  ( 31.03349445238320214, -289.1419799829599810, -239.0131447072785704 ) ) ;
#14097=CARTESIAN_POINT ( 'NONE',  ( 26.81647790735256009, -294.9390734718807039, -230.3493690000086644 ) ) ;
#14099=CARTESIAN_POINT ( 'NONE',  ( -103.6363538570313096, -276.0870243308464183, -305.4327522875097429 ) ) ;
#14100=CARTESIAN_POINT ( 'NONE',  ( -112.4097825472989882, -289.5437952340702168, -286.7605638025282246 ) ) ;
#14101=CARTESIAN_POINT ( 'NONE',  ( -50.63509169451015168, -293.6246332432737631, -342.9539974811273737 ) ) ;
#14102=CARTESIAN_POINT ( 'NONE',  ( -14.13739735806126596, -279.0442022216946611, -200.5735064241824546 ) ) ;
#14103=CARTESIAN_POINT ( 'NONE',  ( -106.7502204742301615, -270.9861988575748342, -243.3160498892666226 ) ) ;
#14104=CARTESIAN_POINT ( 'NONE',  ( -75.24822797616758407, -292.8510157606232269, -207.3387023714448958 ) ) ;
#14105=CARTESIAN_POINT ( 'NONE',  ( -110.4683760289727132, -275.2662352645559167, -253.7030783399848985 ) ) ;
#14106=CARTESIAN_POINT ( 'NONE',  ( -81.48651210148868529, -294.1202050282088862, -332.6666750782173381 ) ) ;
#14107=CARTESIAN_POINT ( 'NONE',  ( -69.08380399028303032, -291.0769227756809414, -336.9860326926581138 ) ) ;
#14108=CARTESIAN_POINT ( 'NONE',  ( -11.47681702660815439, -290.6242242308686059, -198.8566549883668984 ) ) ;
#14109=CARTESIAN_POINT ( 'NONE',  ( 8.359956293620339096, -289.8375919047977050, -328.0389604849112857 ) ) ;
#14112=CARTESIAN_POINT ( 'NONE',  ( -102.9858247835699956, -290.9182363022114828, -302.6636043362885857 ) ) ;
#14113=DIRECTION ( 'NONE',  ( 1.000000000000000000, 0.000000000000000000, 0.000000000000000000 ) ) ;
#14114=CARTESIAN_POINT ( 'NONE',  ( -91.30784694221851794, -291.0037857385912616, -324.8017373036926188 ) ) ;
#14115=CARTESIAN_POINT ( 'NONE',  ( 14.05824733944782778, -278.7890413343747582, -215.1857518931317088 ) ) ;
#14116=CARTESIAN_POINT ( 'NONE',  ( -110.3370467479457488, -290.5412790711283719, -271.1853581452883759 ) ) ;
#14117=CARTESIAN_POINT ( 'NONE',  ( -64.73877283943173211, -280.0374185052302778, -198.3664239154715574 ) ) ;
#14118=CARTESIAN_POINT ( 'NONE',  ( -4.176790403371398064, -282.2935211286444996, -339.8438188120722430 ) ) ;
#14119=CARTESIAN_POINT ( 'NONE',  ( 21.05512804257926973, -286.1996689679367023, -317.4228977309759898 ) ) ;
#14121=CARTESIAN_POINT ( 'NONE',  ( -8.027927935568946793, -280.8035908748170755, -338.5635244063798268 ) ) ;
#14122=CARTESIAN_POINT ( 'NONE',  ( -111.8302403431622025, -282.6642618400067022, -261.6170900516407301 ) ) ;
#14124=CARTESIAN_POINT ( 'NONE',  ( -111.5059496475745817, -276.8047578784135112, -288.3706192000817055 ) ) ;
#14125=CARTESIAN_POINT ( 'NONE',  ( -33.72808386111950085, -285.0169607894292767, -193.7554113558723259 ) ) ;
#14126=CARTESIAN_POINT ( 'NONE',  ( -68.36032304801969417, -274.4368127803882089, -204.0869427637954061 ) ) ;
#14128=CARTESIAN_POINT ( 'NONE',  ( -70.59928159606376141, -293.2061292531759022, -204.4796054605857023 ) ) ;
#14129=CARTESIAN_POINT ( 'NONE',  ( 38.55455174618943914, -277.0945893176096320, -279.6580517081864059 ) ) ;
#14130=CARTESIAN_POINT ( 'NONE',  ( 25.39156730972660370, -275.7325225945671150, -307.7325595295143330 ) ) ;
#14131=CARTESIAN_POINT ( 'NONE',  ( 2.657451776626097661, -296.5163127450852585, -333.8660656586477558 ) ) ;
#14132=CARTESIAN_POINT ( 'NONE',  ( -68.33071209181052552, -291.8229079404740105, -199.8578784062778197 ) ) ;
#14134=CARTESIAN_POINT ( 'NONE',  ( 32.23030895388706796, -280.0158895914046866, -299.9742829114971983 ) ) ;
#14135=CARTESIAN_POINT ( 'NONE',  ( -36.37623622077202867, -291.8972643645329299, -193.3541384934607663 ) ) ;
#14136=CARTESIAN_POINT ( 'NONE',  ( -105.9267909436664894, -289.9541152488866942, -244.5366736721687460 ) ) ;
#14138=CARTESIAN_POINT ( 'NONE',  ( -55.60847405587371384, -293.2871030211031780, -343.1026165646071036 ) ) ;
#14142=CARTESIAN_POINT ( 'NONE',  ( -52.37631430583841308, -291.3621718976091870, -198.8112805608855069 ) ) ;
#14144=CARTESIAN_POINT ( 'NONE',  ( -82.13390479932374433, -275.1952119285919025, -326.4764044574609443 ) ) ;
#14145=CARTESIAN_POINT ( 'NONE',  ( -98.89656482883303568, -296.2230954529638325, -224.4717785838974464 ) ) ;
#14146=CARTESIAN_POINT ( 'NONE',  ( -71.50341313313676039, -284.8091233526311044, -338.8174956199817984 ) ) ;
#14147=CARTESIAN_POINT ( 'NONE',  ( 32.67057204759569089, -287.1114232466391627, -249.6462226227446877 ) ) ;
#14148=CARTESIAN_POINT ( 'NONE',  ( 25.98113282014890757, -277.5856271784311957, -308.0562977641989164 ) ) ;
#14149=CARTESIAN_POINT ( 'NONE',  ( -48.05344700721762052, -293.2090495897617188, -344.2857781626071301 ) ) ;
#14150=CARTESIAN_POINT ( 'NONE',  ( -109.4695407548448571, -298.5282735630041770, -253.7614606591411359 ) ) ;
#14151=CARTESIAN_POINT ( 'NONE',  ( 35.49818444309396881, -274.4708135002339873, -279.7924967494021757 ) ) ;
#14154=CARTESIAN_POINT ( 'NONE',  ( -113.1175540203705623, -296.3884551442629345, -256.8051503496591295 ) ) ;
#14155=CARTESIAN_POINT ( 'NONE',  ( -37.24201843854251592, -290.9710475411726520, -344.8010552855283777 ) ) ;
#14156=CARTESIAN_POINT ( 'NONE',  ( 201.9705131854365447, 295.6986650756944073, -54.00000000004518341 ) ) ;
#14158=CARTESIAN_POINT ( 'NONE',  ( -34.78611012348081033, -299.1631092010823636, -193.6697713408974835 ) ) ;
#14159=CARTESIAN_POINT ( 'NONE',  ( 35.75718393720510591, -288.2123652740634725, -271.0288127003307181 ) ) ;
#14161=CARTESIAN_POINT ( 'NONE',  ( -35.33014468717838241, -279.1355433263214536, -193.6096747170174410 ) ) ;
#14162=CARTESIAN_POINT ( 'NONE',  ( 23.09671377799005398, -294.8404175330675798, -317.9270776544768751 ) ) ;
#14163=CARTESIAN_POINT ( 'NONE',  ( -48.70747715547289403, -287.3348507612859635, -345.3216393609402530 ) ) ;
#14164=CARTESIAN_POINT ( 'NONE',  ( -56.06103340487253206, -295.6201691311474065, -345.0292561213195768 ) ) ;
#14165=CARTESIAN_POINT ( 'NONE',  ( 28.75585337935925168, -293.4648975184543929, -239.2063186195713627 ) ) ;
#14169=CARTESIAN_POINT ( 'NONE',  ( -1.314154478590634278, -288.0413204921113106, -203.0950514380840843 ) ) ;
#14170=CARTESIAN_POINT ( 'NONE',  ( -37.37352853689063181, -286.5523547857346784, -350.3611179825600175 ) ) ;
#14172=EDGE_CURVE ( 'NONE', #17445, #8997, #88492, .T. ) ;
#14173=CARTESIAN_POINT ( 'NONE',  ( -48.09630881610384279, -279.2674814716438050, -194.1650367415545020 ) ) ;
#14174=CARTESIAN_POINT ( 'NONE',  ( -38.89830137828109002, -285.0718496014401921, -345.1910694533187893 ) ) ;
#14176=CARTESIAN_POINT ( 'NONE',  ( -113.7661462205223586, -283.0959919291440769, -272.8120843317425397 ) ) ;
#14177=CARTESIAN_POINT ( 'NONE',  ( -61.74980847409231899, -287.4516782703860827, -340.6857825303348477 ) ) ;
#14178=CARTESIAN_POINT ( 'NONE',  ( -2.022198592863591049, -278.4499099738467294, -337.3897558477009966 ) ) ;
#14180=CARTESIAN_POINT ( 'NONE',  ( 94.54345169680405547, -300.2393862463458731, -197.2883153065869806 ) ) ;
#14182=CARTESIAN_POINT ( 'NONE',  ( -90.96785078138927361, -277.8401073496189611, -319.9647979423762649 ) ) ;
#14183=CARTESIAN_POINT ( 'NONE',  ( -98.07367298108675868, -278.4661649640432870, -229.5831649437682245 ) ) ;
#14184=CARTESIAN_POINT ( 'NONE',  ( -7.822324366002685103, -275.5095474325788700, -199.5227006182154810 ) ) ;
#14185=CARTESIAN_POINT ( 'NONE',  ( -39.56030281678912530, -278.8198367648004705, -193.7773402192825927 ) ) ;
#14186=CARTESIAN_POINT ( 'NONE',  ( -95.74932028542542639, -238.2749555927843232, -339.3703418869641837 ) ) ;
#14187=CARTESIAN_POINT ( 'NONE',  ( -26.33373882931265797, -299.6126883303970203, -193.9477346639631890 ) ) ;
#14188=CARTESIAN_POINT ( 'NONE',  ( -106.6379572354042296, -280.6233781216988064, -303.7686719486574702 ) ) ;
#14190=CARTESIAN_POINT ( 'NONE',  ( 82.65773576150654378, -298.8603700640330203, -192.9535473779746724 ) ) ;
#14191=CARTESIAN_POINT ( 'NONE',  ( -5.677535348280483340, -287.5582457579403126, -204.2291493985908346 ) ) ;
#14192=CARTESIAN_POINT ( 'NONE',  ( -49.20887793360314078, -287.6631892535194197, -195.2538132873395966 ) ) ;
#14193=CARTESIAN_POINT ( 'NONE',  ( 34.38255800710944499, -287.0876648124894928, -284.5510676103588139 ) ) ;
#14194=CARTESIAN_POINT ( 'NONE',  ( -109.9171261506474053, -284.3822664810689957, -244.8202792964235073 ) ) ;
#14195=CARTESIAN_POINT ( 'NONE',  ( -19.31968362216153423, -278.6876171533806428, -198.7425653684849181 ) ) ;
#14196=CARTESIAN_POINT ( 'NONE',  ( -4.061699936632904517, -288.3562535035087535, -204.0036988748265969 ) ) ;
#14197=CARTESIAN_POINT ( 'NONE',  ( 13.83034686957175907, -279.2650493483789091, -217.2604729213304608 ) ) ;
#14198=CARTESIAN_POINT ( 'NONE',  ( -104.7168326204546958, -279.4737261488638751, -299.8455967829389692 ) ) ;
#14199=CARTESIAN_POINT ( 'NONE',  ( 20.88976132196879476, -276.6640622060129999, -314.4869079384255883 ) ) ;
#14200=CARTESIAN_POINT ( 'NONE',  ( -65.31639146576048915, -288.2045816540982628, -341.7293442114217896 ) ) ;
#14201=CARTESIAN_POINT ( 'NONE',  ( -16.17648113013402167, -283.5882415294979637, -344.2823333714444516 ) ) ;
#14202=CARTESIAN_POINT ( 'NONE',  ( -16.15276157233750709, -283.2778061240057355, -344.3795666996779801 ) ) ;
#14203=CARTESIAN_POINT ( 'NONE',  ( -51.82943686677517547, -280.0283971227688653, -198.7614627879414968 ) ) ;
#14204=ORIENTED_EDGE ( 'NONE', *, *, #72721, .T. ) ;
#14207=CARTESIAN_POINT ( 'NONE',  ( -38.87110185356192460, -290.9315582267295213, -346.1104837494446542 ) ) ;
#14208=CARTESIAN_POINT ( 'NONE',  ( -112.6834480584939513, -289.4044036098612196, -257.0600168155260121 ) ) ;
#14209=CARTESIAN_POINT ( 'NONE',  ( -69.58378455677630825, -272.6756725679842930, -204.6050806885176030 ) ) ;
#14210=CARTESIAN_POINT ( 'NONE',  ( 36.98619770398142492, -292.6530194230733741, -250.5954167111473794 ) ) ;
#14211=CARTESIAN_POINT ( 'NONE',  ( -70.29977354516110211, -287.9744968870369348, -336.2877284964466185 ) ) ;
#14212=CARTESIAN_POINT ( 'NONE',  ( 11.61768635659905335, -290.9820608666790349, -214.7863818383469550 ) ) ;
#14213=CARTESIAN_POINT ( 'NONE',  ( 6.091885390431315273, -289.6533626928944614, -329.5907933993488541 ) ) ;
#14214=CARTESIAN_POINT ( 'NONE',  ( -85.28047601435908120, -298.1948066931273615, -330.5268031993605859 ) ) ;
#14216=CARTESIAN_POINT ( 'NONE',  ( 35.56638046930439145, -289.7788260828892817, -288.0055735061279165 ) ) ;
#14217=CARTESIAN_POINT ( 'NONE',  ( -110.1526799126705640, -288.3120511529845658, -289.0832344735468382 ) ) ;
#14218=CARTESIAN_POINT ( 'NONE',  ( -97.86266170161671596, -293.1564090492837522, -226.0427848314624555 ) ) ;
#14219=CARTESIAN_POINT ( 'NONE',  ( -101.2023494514472759, -285.9835899968436479, -234.4071123281624409 ) ) ;
#14220=CARTESIAN_POINT ( 'NONE',  ( -37.80979746801674679, -294.0464577434153739, -195.1959045114138860 ) ) ;
#14223=CARTESIAN_POINT ( 'NONE',  ( -111.4553565240433528, -274.7096953083733979, -256.4595232962145133 ) ) ;
#14224=CARTESIAN_POINT ( 'NONE',  ( 35.29883792459870762, -280.8694551212503825, -279.4885035443959964 ) ) ;
#14225=CARTESIAN_POINT ( 'NONE',  ( -36.18762025512417324, -281.0375223380966645, -345.3522424731692695 ) ) ;
#14226=CARTESIAN_POINT ( 'NONE',  ( -58.81601623219235364, -294.5200876741650973, -344.1933509878840027 ) ) ;
#14227=CARTESIAN_POINT ( 'NONE',  ( 34.49809583749038921, -273.5602740460585665, -252.5561262191338017 ) ) ;
#14228=CARTESIAN_POINT ( 'NONE',  ( -110.9190242024540822, -276.4858121540642060, -281.6611879185322778 ) ) ;
#14229=CARTESIAN_POINT ( 'NONE',  ( -94.84759697801591471, -298.5092289026271146, -224.5974281484274400 ) ) ;
#14232=CARTESIAN_POINT ( 'NONE',  ( 36.20968394733429108, -294.9465510372061772, -268.0012840673191477 ) ) ;
#14234=CARTESIAN_POINT ( 'NONE',  ( -15.53497142895008842, -295.5655699014115498, -340.2504194071890424 ) ) ;
#14236=CARTESIAN_POINT ( 'NONE',  ( 37.04705901611494312, -285.7300419957728081, -282.7076432368932615 ) ) ;
#14237=CARTESIAN_POINT ( 'NONE',  ( -109.3629154386667039, -296.3949860817008357, -282.2751662108620394 ) ) ;
#14238=AXIS2_PLACEMENT_3D ( 'NONE', #44823, #73726, #72790 ) ;
#14239=CARTESIAN_POINT ( 'NONE',  ( -89.88624419584542125, -285.3349789301513511, -214.0029802891857571 ) ) ;
#14240=CARTESIAN_POINT ( 'NONE',  ( 10.21155089039267772, -288.0835995478629457, -330.9634850495824594 ) ) ;
#14241=CARTESIAN_POINT ( 'NONE',  ( -80.89994843296568661, -297.6196557704391239, -331.9153697411414896 ) ) ;
#14242=CARTESIAN_POINT ( 'NONE',  ( 36.29157792888948109, -291.3793049198741869, -256.9417436737648472 ) ) ;
#14243=CARTESIAN_POINT ( 'NONE',  ( -53.71607589525477522, -279.0444812739403915, -195.2331100209836450 ) ) ;
#14244=CARTESIAN_POINT ( 'NONE',  ( -106.6379572354042153, -288.4809262143061801, -236.9535640164627068 ) ) ;
#14246=CARTESIAN_POINT ( 'NONE',  ( 35.67094816608467056, -286.2486388854542270, -262.8588720900862654 ) ) ;
#14248=DIRECTION ( 'NONE',  ( -1.000000000000000000, -0.000000000000000000, -0.000000000000000000 ) ) ;
#14249=CARTESIAN_POINT ( 'NONE',  ( -110.1488601851401086, -297.9948560709354979, -282.4258542162618255 ) ) ;
#14250=CARTESIAN_POINT ( 'NONE',  ( -5.208420572980950070, -281.8921039473032124, -201.0353749997505304 ) ) ;
#14251=CARTESIAN_POINT ( 'NONE',  ( -112.3094908349356587, -294.4747353692621346, -277.9924453798475952 ) ) ;
#14252=CARTESIAN_POINT ( 'NONE',  ( -3.621382056685119366, -282.5941510114553807, -335.1203171167811661 ) ) ;
#14253=CARTESIAN_POINT ( 'NONE',  ( -90.71054468357515077, -295.9501476676332459, -325.9391764204722222 ) ) ;
#14254=CARTESIAN_POINT ( 'NONE',  ( -72.00811300848877750, -299.1051974635101942, -205.3164247607639652 ) ) ;
#14255=CARTESIAN_POINT ( 'NONE',  ( 35.31350075570422575, -285.3648001298708436, -249.4257557264824641 ) ) ;
#14256=CARTESIAN_POINT ( 'NONE',  ( -103.0538490769798727, -281.0330144581539003, -234.2098506933050430 ) ) ;
#14257=CARTESIAN_POINT ( 'NONE',  ( -72.95083854761396935, -296.6266206054201575, -206.3658235504279617 ) ) ;
#14260=CARTESIAN_POINT ( 'NONE',  ( -51.30131951584609595, -285.2112569108211346, -343.7417190541564196 ) ) ;
#14262=CARTESIAN_POINT ( 'NONE',  ( -95.95921662488163406, -288.6952119285919025, -223.5744983911110353 ) ) ;
#14263=CARTESIAN_POINT ( 'NONE',  ( 28.95146154147641226, -275.2560932590581046, -309.2118005502748588 ) ) ;
#14264=CARTESIAN_POINT ( 'NONE',  ( -49.68663578538645709, -291.7237682209976128, -198.3611819217205721 ) ) ;
#14265=CARTESIAN_POINT ( 'NONE',  ( 20.73926454629947003, -283.7055555390929271, -315.7186895342273374 ) ) ;
#14266=CARTESIAN_POINT ( 'NONE',  ( 8.088727632410259716, -278.0196545135936503, -328.5856570530591512 ) ) ;
#14267=CARTESIAN_POINT ( 'NONE',  ( -71.36308232692036313, -285.0940316092591615, -338.5445908440448193 ) ) ;
#14268=CARTESIAN_POINT ( 'NONE',  ( 15.55614868350091484, -279.6157216648200574, -219.4067886766206641 ) ) ;
#14269=CARTESIAN_POINT ( 'NONE',  ( -111.9585651631078349, -280.6559419411130420, -262.2904363817988838 ) ) ;
#14270=CARTESIAN_POINT ( 'NONE',  ( -51.80061419763302411, -297.8721966428390715, -194.6764950348952823 ) ) ;
#14271=CARTESIAN_POINT ( 'NONE',  ( 34.72250017151666412, -275.0423065454774019, -243.2363868378625966 ) ) ;
#14272=CARTESIAN_POINT ( 'NONE',  ( 30.81819672352433059, -295.8671014372986292, -300.2867367104673235 ) ) ;
#14273=DIRECTION ( 'NONE',  ( -1.000000000000000000, -0.000000000000000000, -0.000000000000000000 ) ) ;
#14275=CARTESIAN_POINT ( 'NONE',  ( -37.70718656255608892, -293.1962375127823748, -346.1379083971611408 ) ) ;
#14276=CARTESIAN_POINT ( 'NONE',  ( -1.687124038305205964, -274.0458954562907365, -206.5757981471153357 ) ) ;
#14277=CARTESIAN_POINT ( 'NONE',  ( 25.90726562454861792, -294.5035958607532507, -227.5800757360402145 ) ) ;
#14278=CARTESIAN_POINT ( 'NONE',  ( -61.57757895080220578, -292.9493389620859034, -197.6372970451216702 ) ) ;
#14280=CARTESIAN_POINT ( 'NONE',  ( -53.78724688457625547, -291.2638794748968962, -343.3650385295980527 ) ) ;
#14281=CARTESIAN_POINT ( 'NONE',  ( -94.13420992225614725, -275.8752571882094458, -319.0913884559705025 ) ) ;
#14283=CARTESIAN_POINT ( 'NONE',  ( -39.16907858581424762, -278.9954182093110830, -344.7786890849434940 ) ) ;
#14284=CARTESIAN_POINT ( 'NONE',  ( 34.01635981290764477, -291.3548121382031582, -248.9856146860099955 ) ) ;
#14285=CARTESIAN_POINT ( 'NONE',  ( 29.99044357938772620, -283.8676159804514327, -305.0985315538025588 ) ) ;
#14286=CARTESIAN_POINT ( 'NONE',  ( -108.9639664917576170, -283.6786396429121169, -254.6667992937428551 ) ) ;
#14288=CARTESIAN_POINT ( 'NONE',  ( -84.87875752425213705, -283.3961050905382422, -325.7895913585948620 ) ) ;
#14289=CARTESIAN_POINT ( 'NONE',  ( -86.61667922215481497, -280.4658425669377380, -211.5256669765586821 ) ) ;
#14291=CARTESIAN_POINT ( 'NONE',  ( -89.60407103446807753, -284.1300972530459603, -214.2831545936875557 ) ) ;
#14293=CARTESIAN_POINT ( 'NONE',  ( -114.1426543907955846, -279.5135989684816877, -268.7511795043266716 ) ) ;
#14294=CARTESIAN_POINT ( 'NONE',  ( -31.48399781683347598, -278.4997139785344871, -346.4947700724522974 ) ) ;
#14295=CARTESIAN_POINT ( 'NONE',  ( 7.399455738971494334, -295.1948066931273615, -214.2051214447836571 ) ) ;
#14296=VERTEX_POINT ( 'NONE', #24557 ) ;
#14297=CARTESIAN_POINT ( 'NONE',  ( -37.86125051787408324, -300.0458004373203380, -195.3629131990695100 ) ) ;
#14299=CARTESIAN_POINT ( 'NONE',  ( -84.05530198637387684, -275.7174392797251130, -328.6486712496747487 ) ) ;
#14300=CARTESIAN_POINT ( 'NONE',  ( -93.97127794204811835, -293.0086743298103329, -219.6949070399757034 ) ) ;
#14301=CARTESIAN_POINT ( 'NONE',  ( 33.54287338358038539, -293.1362273302929680, -288.2292434180315013 ) ) ;
#14302=CARTESIAN_POINT ( 'NONE',  ( -98.98359706906708766, -289.4465440357764692, -316.4242299082336558 ) ) ;
#14304=CARTESIAN_POINT ( 'NONE',  ( 33.89555699529996247, -292.4797392001759135, -297.9991260371943440 ) ) ;
#14305=CARTESIAN_POINT ( 'NONE',  ( -39.98235887477027006, -284.4182903699092435, -196.6083733684679373 ) ) ;
#14306=CARTESIAN_POINT ( 'NONE',  ( -82.49888445813341775, -293.2888127168125720, -211.3749697095003341 ) ) ;
#14307=CARTESIAN_POINT ( 'NONE',  ( -37.52504634485897128, -284.3697058703475591, -343.8665548960725573 ) ) ;
#14308=CARTESIAN_POINT ( 'NONE',  ( -67.94901620420786514, -290.3855031714980441, -340.7600697937497216 ) ) ;
#14309=CARTESIAN_POINT ( 'NONE',  ( 15.29937166111044178, -281.3128708793848887, -219.6242090191550176 ) ) ;
#14310=CARTESIAN_POINT ( 'NONE',  ( 37.67859556694827461, -292.5418195981741292, -285.8518879379860778 ) ) ;
#14312=CARTESIAN_POINT ( 'NONE',  ( -57.23920504870751103, -290.1052557830640808, -344.6336781534574243 ) ) ;
#14313=CARTESIAN_POINT ( 'NONE',  ( -114.0505846474586633, -290.9619720733787176, -276.9545647009172171 ) ) ;
#14314=CARTESIAN_POINT ( 'NONE',  ( -99.61042734543107713, -285.2449734497383815, -232.1648608034618348 ) ) ;
#14317=CARTESIAN_POINT ( 'NONE',  ( 35.90853383186513526, -295.6588484749536292, -289.7185121165886130 ) ) ;
#14318=CARTESIAN_POINT ( 'NONE',  ( -69.33704263861280026, -294.1492102889079661, -339.8707575857851566 ) ) ;
#14319=CARTESIAN_POINT ( 'NONE',  ( -85.63036447662732087, -278.4230117712170909, -215.3010295072877796 ) ) ;
#14320=CARTESIAN_POINT ( 'NONE',  ( -111.7571421343270828, -272.3069483100372281, -250.6158138224584491 ) ) ;
#14321=CARTESIAN_POINT ( 'NONE',  ( -53.31837622300675861, -293.7405077996714908, -342.3542243935117426 ) ) ;
#14322=CARTESIAN_POINT ( 'NONE',  ( 28.94793848021655336, -277.7538982752317338, -303.3956843138654449 ) ) ;
#14323=CARTESIAN_POINT ( 'NONE',  ( -88.16193199841627859, -271.4716836609904362, -216.1781961916792341 ) ) ;
#14324=CARTESIAN_POINT ( 'NONE',  ( 23.66279123890370784, -294.1935082302219371, -229.5495689064723877 ) ) ;
#14325=CARTESIAN_POINT ( 'NONE',  ( -38.33273780458437585, -296.1445374993913333, -343.6635321238021561 ) ) ;
#14327=CARTESIAN_POINT ( 'NONE',  ( -98.41669451788361300, -295.1468274297305925, -226.5447570133376871 ) ) ;
#14328=CARTESIAN_POINT ( 'NONE',  ( -110.8855674913601916, -273.6370343332343964, -247.9202626443962174 ) ) ;
#14329=CARTESIAN_POINT ( 'NONE',  ( -71.46195304328433906, -288.0867280163058126, -335.5764546452123227 ) ) ;
#14330=CARTESIAN_POINT ( 'NONE',  ( -70.39471015352404493, -275.6166088412659292, -203.0372798450532059 ) ) ;
#14331=CARTESIAN_POINT ( 'NONE',  ( -80.53665008232570699, -290.5949559425654911, -329.5647661375521125 ) ) ;
#14332=CARTESIAN_POINT ( 'NONE',  ( -102.6700982655681145, -273.5766017732141222, -229.7196699284725980 ) ) ;
#14333=CARTESIAN_POINT ( 'NONE',  ( -36.99118546351476056, -295.3808934616963029, -343.3938486620118056 ) ) ;
#14334=CARTESIAN_POINT ( 'NONE',  ( -100.7000855771482719, -279.9839943951257055, -311.2499353221423348 ) ) ;
#14335=CARTESIAN_POINT ( 'NONE',  ( 36.85710487862867524, -280.0021296299444202, -251.7107665126004861 ) ) ;
#14337=CARTESIAN_POINT ( 'NONE',  ( -83.82819128536965536, -283.0199325487519104, -331.6841877645991303 ) ) ;
#14338=CARTESIAN_POINT ( 'NONE',  ( 28.41968782960035966, -274.3786126869667896, -230.4001445614988768 ) ) ;
#14339=CARTESIAN_POINT ( 'NONE',  ( -95.28408749624401253, -277.6267714759453611, -220.8524973914401528 ) ) ;
#14340=CARTESIAN_POINT ( 'NONE',  ( -6.947759595097298124, -278.4498802102265245, -201.5995516875902354 ) ) ;
#14341=CARTESIAN_POINT ( 'NONE',  ( -93.10774604524576148, -295.9140532030214672, -222.4732841039282221 ) ) ;
#14342=CARTESIAN_POINT ( 'NONE',  ( 10.71227879108921677, -278.3885824922330698, -328.0110159857105714 ) ) ;
#14344=CARTESIAN_POINT ( 'NONE',  ( -67.64371597904676037, -289.6766827145651746, -201.3528966301584830 ) ) ;
#14345=CARTESIAN_POINT ( 'NONE',  ( -34.96041325354462259, -292.0812526684684940, -193.3847983342242856 ) ) ;
#14346=CARTESIAN_POINT ( 'NONE',  ( -62.95685507476765963, -275.7195489670623374, -199.6936412841522497 ) ) ;
#14347=CARTESIAN_POINT ( 'NONE',  ( -33.67497888491850233, -296.0979968831556448, -195.5290295220289636 ) ) ;
#14348=CARTESIAN_POINT ( 'NONE',  ( -57.70328141361187591, -284.9930276645395679, -196.2142869132435692 ) ) ;
#14350=CARTESIAN_POINT ( 'NONE',  ( -105.2991944055074640, -282.1335462649419696, -302.2120066413933159 ) ) ;
#14352=CARTESIAN_POINT ( 'NONE',  ( -7.092655917093349416, -291.2530438912422710, -203.4871631851719087 ) ) ;
#14353=CARTESIAN_POINT ( 'NONE',  ( -33.14553820353298619, -284.2449980680555655, -196.1939413430673085 ) ) ;
#14356=CARTESIAN_POINT ( 'NONE',  ( 9.456786886954839488, -292.4090604644089240, -329.0358840124710014 ) ) ;
#14357=CARTESIAN_POINT ( 'NONE',  ( -110.2577045908584097, -283.3191233880940558, -247.6897766699752310 ) ) ;
#14358=CARTESIAN_POINT ( 'NONE',  ( -109.3921927708529154, -280.3614092548899634, -254.3292481511692529 ) ) ;
#14359=CARTESIAN_POINT ( 'NONE',  ( -111.4867405742397608, -285.5144640518292931, -289.6620207348321969 ) ) ;
#14360=CARTESIAN_POINT ( 'NONE',  ( 9.030491218528814201, -286.7095643496063531, -213.9818676353500564 ) ) ;
#14362=CARTESIAN_POINT ( 'NONE',  ( -108.3844002298262552, -279.7259553979386624, -289.5525139859456090 ) ) ;
#14363=CARTESIAN_POINT ( 'NONE',  ( -109.2927588218234973, -279.5294332073900705, -257.1079342077688352 ) ) ;
#14364=CARTESIAN_POINT ( 'NONE',  ( -2.995578734438594459, -288.4835234001902791, -203.2739552042093862 ) ) ;
#14366=CARTESIAN_POINT ( 'NONE',  ( -106.5123895386246602, -296.8198847725601013, -236.5319038185529621 ) ) ;
#14367=CARTESIAN_POINT ( 'NONE',  ( 28.49276693186321197, -290.0023076678758684, -305.6517272371286822 ) ) ;
#14369=CARTESIAN_POINT ( 'NONE',  ( -111.2586520408596868, -280.6233781216988064, -305.9938812882205070 ) ) ;
#14371=CARTESIAN_POINT ( 'NONE',  ( -69.32790274241071415, -271.6322069536284971, -202.3256464850647092 ) ) ;
#14372=CARTESIAN_POINT ( 'NONE',  ( 24.18072300293407650, -291.3488767565308422, -225.4007813636752076 ) ) ;
#14373=CARTESIAN_POINT ( 'NONE',  ( 35.96210039831592553, -288.9733974347189474, -262.7940458914929991 ) ) ;
#14375=CARTESIAN_POINT ( 'NONE',  ( -5.137559053294268985, -282.2421465115551200, -203.7212851917494447 ) ) ;
#14376=CARTESIAN_POINT ( 'NONE',  ( 19.20054947509118648, -289.6814480229082847, -321.7769188502545035 ) ) ;
#14377=CARTESIAN_POINT ( 'NONE',  ( 12.10990499644116447, -289.6959510529090380, -328.7378001602225481 ) ) ;
#14378=CARTESIAN_POINT ( 'NONE',  ( -102.1159769201279914, -286.0472506377767559, -308.1671189971334002 ) ) ;
#14379=CARTESIAN_POINT ( 'NONE',  ( -106.1765300566876249, -279.1640474096077469, -235.7348802015663409 ) ) ;
#14381=CARTESIAN_POINT ( 'NONE',  ( -53.01488439969033806, -293.3312470911025684, -344.3312566764533358 ) ) ;
#14382=CARTESIAN_POINT ( 'NONE',  ( 21.97206431031955987, -280.7254256191153559, -221.2604321148812687 ) ) ;
#14383=CARTESIAN_POINT ( 'NONE',  ( -95.59651220086031742, -275.0510408405118596, -224.3476161127082094 ) ) ;
#14385=CARTESIAN_POINT ( 'NONE',  ( 39.58706461736021254, -284.0519495502703080, -270.3284710469133074 ) ) ;
#14386=CARTESIAN_POINT ( 'NONE',  ( -0.5166361833813898352, -272.7744315635289922, -203.8791200527144838 ) ) ;
#14388=CARTESIAN_POINT ( 'NONE',  ( -83.47174265841594831, -278.9077171624493303, -213.6387119751212538 ) ) ;
#14389=CARTESIAN_POINT ( 'NONE',  ( 39.23352203135741689, -276.7313282288343999, -268.3010042182835377 ) ) ;
#14390=CARTESIAN_POINT ( 'NONE',  ( -88.54869008841748723, -298.7424631669939572, -217.4390427315784962 ) ) ;
#14391=CARTESIAN_POINT ( 'NONE',  ( -105.5804996657635115, -283.1550370772400242, -305.6379988849880078 ) ) ;
#14392=CARTESIAN_POINT ( 'NONE',  ( -111.3500630253088133, -292.3011370378496849, -271.2191577044074506 ) ) ;
#14393=CARTESIAN_POINT ( 'NONE',  ( -5.467654576524973997, -276.0646365443609511, -201.1477837311212795 ) ) ;
#14394=CARTESIAN_POINT ( 'NONE',  ( 19.00999114233902532, -299.9479996367310832, -193.7469286884922042 ) ) ;
#14395=CARTESIAN_POINT ( 'NONE',  ( 37.11684435756603051, -295.4496335706466539, -262.3817342449729040 ) ) ;
#14396=CARTESIAN_POINT ( 'NONE',  ( -23.75706508060757116, -280.8779958869529878, -343.9511044907413293 ) ) ;
#14397=CARTESIAN_POINT ( 'NONE',  ( -69.61042414466034245, -291.3056377119316949, -200.4577705646783841 ) ) ;
#14398=CARTESIAN_POINT ( 'NONE',  ( 3.858336639969510262, -272.6295016965917171, -208.0546229927558670 ) ) ;
#14399=CARTESIAN_POINT ( 'NONE',  ( 1.100306331594340881, -288.1564328317358559, -204.5534449166346178 ) ) ;
#14400=CARTESIAN_POINT ( 'NONE',  ( -67.91763419731228169, -290.5614137982711327, -203.7189671608931292 ) ) ;
#14401=ORIENTED_EDGE ( 'NONE', *, *, #77244, .T. ) ;
#14402=CARTESIAN_POINT ( 'NONE',  ( -98.56797433984831969, -288.5137697662556775, -316.0987284368306973 ) ) ;
#14403=CARTESIAN_POINT ( 'NONE',  ( -72.37273330338734922, -289.1961088348058411, -334.4307223319834748 ) ) ;
#14405=CARTESIAN_POINT ( 'NONE',  ( -26.67774481461488989, -287.2643021460505679, -194.3619817108954919 ) ) ;
#14406=CARTESIAN_POINT ( 'NONE',  ( -21.64434047212760603, -277.1787543336715771, -341.7270826073668673 ) ) ;
#14408=CARTESIAN_POINT ( 'NONE',  ( 17.27914756733905222, -291.7295190458441425, -216.4527339613252650 ) ) ;
#14409=CARTESIAN_POINT ( 'NONE',  ( -106.9098968270767784, -284.7833055188969524, -303.1266302526114487 ) ) ;
#14410=CARTESIAN_POINT ( 'NONE',  ( -105.4153796666955998, -285.3508834839694259, -234.3064888435326054 ) ) ;
#14411=CARTESIAN_POINT ( 'NONE',  ( -57.12301384900006695, -280.1230906920644088, -200.0703852067081812 ) ) ;
#14412=CARTESIAN_POINT ( 'NONE',  ( -30.89368022450710427, -124.4715039767320945, -364.4326362608330214 ) ) ;
#14413=B_SPLINE_CURVE_WITH_KNOTS ( 'NONE', 3,
 ( #44914, #74752, #1843, #16982, #31659, #75216, #88478, #52492, #36903, #1377, #38278, #73817, #60091, #88930, #80441, #65820, #52954, #928, #15586, #80916, #58689, #2778, #81832, #22680, #29808, #16061, #67652, #81367 ),
 .UNSPECIFIED., .F., .F.,
 ( 4, 2, 2, 2, 2, 2, 2, 2, 2, 2, 2, 2, 2, 4 ),
 ( 0.0002500661914413574642, 0.001032049840278917571, 0.001423041664697730991, 0.001814033489116544410, 0.002205025313535357613, 0.002596017137954171033, 0.002987008962372984452, 0.003378000786791797872, 0.003768992611210611292, 0.004159984435629425145, 0.004550976260048238999, 0.004941968084467051985, 0.005723951733304678824, 0.006505935382142305663 ),
 .UNSPECIFIED. ) ;
#14414=CARTESIAN_POINT ( 'NONE',  ( -110.7704075034332334, -265.7311065234434295, -306.6539985541684814 ) ) ;
#14415=CARTESIAN_POINT ( 'NONE',  ( -78.21339102487489470, -207.4003955205593286, -353.8744156467298581 ) ) ;
#14416=CARTESIAN_POINT ( 'NONE',  ( -76.64237422815001821, -272.7084510478538846, -208.6516475419634844 ) ) ;
#14417=CARTESIAN_POINT ( 'NONE',  ( 28.14355019523062751, -274.0271315257626270, -237.4079988169975763 ) ) ;
#14418=CARTESIAN_POINT ( 'NONE',  ( -86.36093546960420042, -295.2195732113673330, -329.6623951154217593 ) ) ;
#14419=CARTESIAN_POINT ( 'NONE',  ( 122.4157943089394536, 147.2165473011896495, -260.6027802525132415 ) ) ;
#14420=CARTESIAN_POINT ( 'NONE',  ( -68.62698462865486704, -272.3343739459812127, -200.5289876915827563 ) ) ;
#14421=CARTESIAN_POINT ( 'NONE',  ( -97.90392683170983901, -299.0020315989928577, -227.4299850107997543 ) ) ;
#14422=CARTESIAN_POINT ( 'NONE',  ( -45.39999920894819496, -290.4715657419280888, -343.4111507927168532 ) ) ;
#14423=ORIENTED_EDGE ( 'NONE', *, *, #1254, .T. ) ;
#14424=CARTESIAN_POINT ( 'NONE',  ( -113.4177797433905539, -297.3598249662886133, -281.0091380986908121 ) ) ;
#14425=CARTESIAN_POINT ( 'NONE',  ( -8.236189382415831872, -286.9362470003823660, -203.3472560879000355 ) ) ;
#14426=CARTESIAN_POINT ( 'NONE',  ( -113.2363566762648190, -271.6154328043098758, -258.9769401050100441 ) ) ;
#14427=CARTESIAN_POINT ( 'NONE',  ( -5.854503303691197758, -295.4514383460938234, -340.4518824039713536 ) ) ;
#14428=CARTESIAN_POINT ( 'NONE',  ( -69.49648416890707381, -295.9564390758707759, -340.2725829551996526 ) ) ;
#14430=CARTESIAN_POINT ( 'NONE',  ( -107.7524471625724232, -290.9734253673448166, -251.0912786846745632 ) ) ;
#14432=CARTESIAN_POINT ( 'NONE',  ( -64.40754221795538115, -275.6218271742444017, -199.8010802476034655 ) ) ;
#14433=CARTESIAN_POINT ( 'NONE',  ( 38.74132893143520562, -274.4646653277582686, -279.7147224443534128 ) ) ;
#14435=CARTESIAN_POINT ( 'NONE',  ( -113.6552355532110141, -278.1873650746439353, -260.1697941800567264 ) ) ;
#14436=CARTESIAN_POINT ( 'NONE',  ( 34.29055085857213925, -273.7202609980390662, -252.6055263040511534 ) ) ;
#14437=CARTESIAN_POINT ( 'NONE',  ( -99.55002201677775986, -274.1648812949173362, -231.5751571062340872 ) ) ;
#14438=CARTESIAN_POINT ( 'NONE',  ( 29.37353015692898595, -276.8992233874094495, -300.5685093861888504 ) ) ;
#14439=CARTESIAN_POINT ( 'NONE',  ( 27.62439283027330816, -276.7897786167992535, -230.8476234467975132 ) ) ;
#14440=CARTESIAN_POINT ( 'NONE',  ( 22.20251835274090269, -274.2026633635754820, -316.5652897589919803 ) ) ;
#14441=CARTESIAN_POINT ( 'NONE',  ( -9.183961762373082038, -295.3254441350799198, -337.8360987497922565 ) ) ;
#14442=CARTESIAN_POINT ( 'NONE',  ( 18.04659286505167870, -300.6605412952987990, -194.7831514931514505 ) ) ;
#14443=CARTESIAN_POINT ( 'NONE',  ( 20.14275556054300154, -292.7709200658823647, -316.3258645102907849 ) ) ;
#14445=CARTESIAN_POINT ( 'NONE',  ( -112.4229776781453580, -278.8341882431408862, -287.1637566155142736 ) ) ;
#14446=CARTESIAN_POINT ( 'NONE',  ( -69.24949975702652694, -277.6506388362375901, -336.0323408013662174 ) ) ;
#14447=CIRCLE ( 'NONE', #6870, 6.151811579824029153 ) ;
#14448=CARTESIAN_POINT ( 'NONE',  ( -30.90852138100013491, -284.8166476387335706, -194.1120080189415376 ) ) ;
#14449=CARTESIAN_POINT ( 'NONE',  ( -78.45245292563932082, -297.6042968919602458, -333.2891278769662904 ) ) ;
#14451=CARTESIAN_POINT ( 'NONE',  ( 34.91709743725075299, -286.9011723239887601, -281.8981062075125692 ) ) ;
#14452=CARTESIAN_POINT ( 'NONE',  ( -72.15030934911615645, -275.7589682696256546, -335.6926008550572078 ) ) ;
#14453=CARTESIAN_POINT ( 'NONE',  ( -32.39896772593964869, -275.5634787360673386, -343.8345382929208540 ) ) ;
#14454=CARTESIAN_POINT ( 'NONE',  ( -94.86477220922611764, -285.8871905615400806, -318.5065006035287070 ) ) ;
#14455=CARTESIAN_POINT ( 'NONE',  ( -69.41112767921349302, -278.6888663787347014, -336.3953466727637078 ) ) ;
#14457=CARTESIAN_POINT ( 'NONE',  ( 19.26906676728643930, -274.6518835703760146, -321.3871235923590461 ) ) ;
#14458=CARTESIAN_POINT ( 'NONE',  ( 34.26608482253153909, -276.3972716120188693, -285.0654643800544932 ) ) ;
#14459=CARTESIAN_POINT ( 'NONE',  ( 37.87572481208437125, -283.5466024402552421, -269.9151042571986636 ) ) ;
#14461=CARTESIAN_POINT ( 'NONE',  ( 35.29991974877142269, -289.2044881254864208, -249.3786929451851506 ) ) ;
#14462=CARTESIAN_POINT ( 'NONE',  ( 35.88369702992221733, -291.7609199512125997, -286.6376608965923651 ) ) ;
#14464=CARTESIAN_POINT ( 'NONE',  ( -109.6115687996755668, -271.4155068255307128, -256.7359658464415588 ) ) ;
#14465=CARTESIAN_POINT ( 'NONE',  ( -6.739775739704214175, -290.5978096821435770, -202.7268980437074219 ) ) ;
#14466=CARTESIAN_POINT ( 'NONE',  ( -45.58595926748305516, -157.7977398304416283, -369.2266198007532125 ) ) ;
#14468=CARTESIAN_POINT ( 'NONE',  ( -110.8790282293439873, -288.7745052077437435, -290.7319090694129500 ) ) ;
#14469=CARTESIAN_POINT ( 'NONE',  ( -111.2390156027235832, -282.5670511337223161, -288.1126141131154554 ) ) ;
#14470=CARTESIAN_POINT ( 'NONE',  ( -48.39945455645703731, -284.6209385630046427, -343.1148188022164049 ) ) ;
#14471=CARTESIAN_POINT ( 'NONE',  ( -110.3901388725797545, -285.4194407378547567, -265.4645607995058754 ) ) ;
#14472=CARTESIAN_POINT ( 'NONE',  ( -108.8776233533928774, -292.8385630391066456, -246.5118268269977762 ) ) ;
#14473=CARTESIAN_POINT ( 'NONE',  ( 1.181162909312186704, -274.8851213153484423, -203.6995074189279649 ) ) ;
#14474=CARTESIAN_POINT ( 'NONE',  ( -110.5924412669333066, -288.8689748160747968, -251.7714571291788559 ) ) ;
#14475=CARTESIAN_POINT ( 'NONE',  ( -1.467729270677221587, -276.5897947753927610, -338.4937695889823885 ) ) ;
#14476=CARTESIAN_POINT ( 'NONE',  ( 33.92449846294908156, -295.8197783759478057, -292.5641750120211100 ) ) ;
#14478=CARTESIAN_POINT ( 'NONE',  ( -69.91165696735023971, -300.1233781216987495, -202.8022627189028810 ) ) ;
#14479=CARTESIAN_POINT ( 'NONE',  ( -109.4666706674200043, -283.0520246209561606, -284.4760782690611904 ) ) ;
#14480=CARTESIAN_POINT ( 'NONE',  ( -40.88767294294499521, -278.0074011142497170, -195.4321337789455697 ) ) ;
#14481=CARTESIAN_POINT ( 'NONE',  ( -83.14828806871129530, -271.9179320463293266, -209.2666095534543160 ) ) ;
#14482=CARTESIAN_POINT ( 'NONE',  ( 20.09741051231208431, -275.5379207833321971, -315.5989837358765726 ) ) ;
#14483=CARTESIAN_POINT ( 'NONE',  ( 32.45148768063754119, -294.7590373082715018, -246.5461308311271011 ) ) ;
#14484=CARTESIAN_POINT ( 'NONE',  ( 31.04383635395285168, -294.1445138563373689, -244.1537364318259904 ) ) ;
#14485=CARTESIAN_POINT ( 'NONE',  ( 21.00250380493349667, -295.5386938346554757, -319.8510375773423107 ) ) ;
#14486=CARTESIAN_POINT ( 'NONE',  ( -109.7359493454813872, -296.5143073771769195, -260.5946354563778300 ) ) ;
#14487=CARTESIAN_POINT ( 'NONE',  ( -67.09976804096399405, -291.4422528946016655, -339.2603257240036214 ) ) ;
#14488=CARTESIAN_POINT ( 'NONE',  ( -44.41710106374254252, -283.3058588170700887, -347.0887129046465134 ) ) ;
#14489=CARTESIAN_POINT ( 'NONE',  ( -0.6229824058376443041, -272.6741730467479101, -204.0738858503770530 ) ) ;
#14490=CARTESIAN_POINT ( 'NONE',  ( 28.69963864912850582, -286.8679842640183892, -230.6660903507437581 ) ) ;
#14491=CARTESIAN_POINT ( 'NONE',  ( -100.5548726351711792, -279.9947660874887561, -310.1557495517070038 ) ) ;
#14492=ADVANCED_FACE ( 'NONE', ( #8488 ), #71742, .T. ) ;
#14493=CARTESIAN_POINT ( 'NONE',  ( -11.92913331271559763, -285.4499891673439151, -201.6762586907419745 ) ) ;
#14494=CARTESIAN_POINT ( 'NONE',  ( -38.90471179144449820, -287.0716063474030193, -345.3448338609537700 ) ) ;
#14495=CARTESIAN_POINT ( 'NONE',  ( -111.2639016180397959, -258.5489101121608542, -316.4159311957783984 ) ) ;
#14496=CARTESIAN_POINT ( 'NONE',  ( -109.9346344960164572, -283.9451533273092423, -279.0594627419676499 ) ) ;
#14497=CARTESIAN_POINT ( 'NONE',  ( 25.94386595009920526, -282.1839297177074286, -227.1067327960679165 ) ) ;
#14498=LINE ( 'NONE', #79543, #33699 ) ;
#14499=CARTESIAN_POINT ( 'NONE',  ( -91.44124123220973388, -288.8578038866108386, -324.8974508624912687 ) ) ;
#14500=CARTESIAN_POINT ( 'NONE',  ( -112.9696262617293598, -280.0292301366362722, -280.0977042042364360 ) ) ;
#14501=CARTESIAN_POINT ( 'NONE',  ( -88.61344510260813934, -280.6655455610133458, -213.5763802541279404 ) ) ;
#14502=CARTESIAN_POINT ( 'NONE',  ( -30.26027235691184458, -279.9774076899155943, -197.6550446580477853 ) ) ;
#14503=CARTESIAN_POINT ( 'NONE',  ( -0.9421106629741500260, -276.5177356394447088, -205.1781124975804289 ) ) ;
#14504=CARTESIAN_POINT ( 'NONE',  ( 39.65600365699447138, -293.5155770713311654, -267.4366029175038761 ) ) ;
#14505=CARTESIAN_POINT ( 'NONE',  ( 33.87545233411397305, -285.8640835243630818, -292.8928352280831291 ) ) ;
#14507=CARTESIAN_POINT ( 'NONE',  ( -22.37111331057360530, -293.8407550719356323, -195.5924208132926196 ) ) ;
#14508=CARTESIAN_POINT ( 'NONE',  ( -95.02514531090415062, -294.8372273175374403, -315.6032026661418968 ) ) ;
#14509=CARTESIAN_POINT ( 'NONE',  ( -43.01880810896771123, -285.0443870198723175, -344.6354010910411034 ) ) ;
#14510=CARTESIAN_POINT ( 'NONE',  ( -58.41839577875898470, -294.9989764767250904, -340.2743526892491559 ) ) ;
#14511=CARTESIAN_POINT ( 'NONE',  ( -98.96445349272538294, -292.2413836795672637, -224.6868547161107017 ) ) ;
#14512=CARTESIAN_POINT ( 'NONE',  ( 31.16292369346579960, -281.8619956701181195, -244.7010563432375250 ) ) ;
#14514=CARTESIAN_POINT ( 'NONE',  ( -78.70465440538337987, -272.5681629685304301, -205.6933035302457995 ) ) ;
#14515=CARTESIAN_POINT ( 'NONE',  ( -82.78572066212326774, -290.3070029441332167, -332.3946071959687742 ) ) ;
#14516=CARTESIAN_POINT ( 'NONE',  ( -91.56651892380735092, -281.9541073794486579, -323.2759033108702624 ) ) ;
#14517=CARTESIAN_POINT ( 'NONE',  ( -98.33411376711671892, -291.5125114057701126, -223.3752286448122391 ) ) ;
#14518=CARTESIAN_POINT ( 'NONE',  ( 22.00628498951112633, -287.2899505504071271, -227.7329077464494844 ) ) ;
#14519=CARTESIAN_POINT ( 'NONE',  ( 128.9467878515196162, -299.5541904835127980, -189.1116627405232578 ) ) ;
#14520=CARTESIAN_POINT ( 'NONE',  ( -49.41460023398800416, -154.1821796365580894, -362.9324954162679546 ) ) ;
#14521=CARTESIAN_POINT ( 'NONE',  ( -88.81474777452721980, -229.3358420801235695, -344.3332919790561277 ) ) ;
#14522=CARTESIAN_POINT ( 'NONE',  ( -109.7802148314754760, -277.8889832527767112, -259.7501468087731382 ) ) ;
#14523=CARTESIAN_POINT ( 'NONE',  ( -101.0737859873117941, -277.9665651670258626, -234.1334033853535175 ) ) ;
#14524=CARTESIAN_POINT ( 'NONE',  ( 11.77546588010454798, -274.3792707720593285, -211.0191881301796286 ) ) ;
#14525=CARTESIAN_POINT ( 'NONE',  ( -104.5657734472104181, -261.9804595554911657, -316.2884981726831484 ) ) ;
#14526=CARTESIAN_POINT ( 'NONE',  ( -111.5095649910323203, -277.3591769470508552, -251.9299453443525465 ) ) ;
#14527=CARTESIAN_POINT ( 'NONE',  ( -92.90589819667893323, -281.8744731503331877, -320.2247838378879692 ) ) ;
#14528=CARTESIAN_POINT ( 'NONE',  ( -113.2204528967522918, -298.2497500708282701, -275.2961954638095676 ) ) ;
#14529=CARTESIAN_POINT ( 'NONE',  ( -104.7622770194931690, -291.4233665442075676, -242.0788721421332639 ) ) ;
#14530=CARTESIAN_POINT ( 'NONE',  ( -56.20823887814563591, -287.9850105642919402, -341.4442886955926610 ) ) ;
#14531=CARTESIAN_POINT ( 'NONE',  ( 9.441750169202579812, -275.3279548545359603, -209.3314402466088495 ) ) ;
#14532=CARTESIAN_POINT ( 'NONE',  ( -62.02969541815978971, -273.7220155636430832, -201.6624797969521126 ) ) ;
#14536=CARTESIAN_POINT ( 'NONE',  ( -100.6974140603196304, -281.0244191217836374, -229.0915537689155030 ) ) ;
#14537=CARTESIAN_POINT ( 'NONE',  ( -6.652513635218989307, -281.5444808028910870, -203.7711441255180773 ) ) ;
#14538=CARTESIAN_POINT ( 'NONE',  ( 16.48920718330317214, -282.5641733604166461, -216.6570758301816682 ) ) ;
#14539=CARTESIAN_POINT ( 'NONE',  ( -64.15263536178552783, -282.4694777003194872, -338.5122896539165822 ) ) ;
#14540=CARTESIAN_POINT ( 'NONE',  ( -100.2087378817642644, -279.8753090915332677, -309.9362131319967943 ) ) ;
#14541=CARTESIAN_POINT ( 'NONE',  ( -32.62752405860703675, -272.5924860293567917, -196.8060748556924864 ) ) ;
#14544=CARTESIAN_POINT ( 'NONE',  ( -111.2823407084260907, -279.0924499792002393, -291.2642395510175106 ) ) ;
#14546=CARTESIAN_POINT ( 'NONE',  ( -20.27550205217131563, -275.4119303759320019, -344.8959571593156284 ) ) ;
#14547=ORIENTED_EDGE ( 'NONE', *, *, #89262, .T. ) ;
#14549=CARTESIAN_POINT ( 'NONE',  ( -63.32079117999034423, -285.3688541233674982, -341.0964954846953674 ) ) ;
#14550=CARTESIAN_POINT ( 'NONE',  ( 33.80719320609994583, -292.5243391545574241, -253.2653617537477544 ) ) ;
#14551=CARTESIAN_POINT ( 'NONE',  ( -54.48697109193350485, -288.6153082511057164, -345.3780989725769928 ) ) ;
#14552=CARTESIAN_POINT ( 'NONE',  ( -110.5034815241817796, -282.6420615652609172, -281.8855572341871607 ) ) ;
#14553=CARTESIAN_POINT ( 'NONE',  ( -110.5789524541091282, -283.2275121335682684, -262.6705760848790305 ) ) ;
#14554=CARTESIAN_POINT ( 'NONE',  ( 24.74842285157107824, -285.0722433439945007, -229.2052258075054283 ) ) ;
#14555=CARTESIAN_POINT ( 'NONE',  ( -3.424320888788228601, -283.7990318890963408, -335.4654600628635990 ) ) ;
#14556=CARTESIAN_POINT ( 'NONE',  ( -27.24000820384891952, -272.1802448852197358, -195.9924783395721590 ) ) ;
#14557=CARTESIAN_POINT ( 'NONE',  ( -75.68634411076639879, -283.9496400395147475, -204.4510765533989343 ) ) ;
#14558=CARTESIAN_POINT ( 'NONE',  ( -34.89372829054680381, -297.0215532170644224, -345.3211612423731367 ) ) ;
#14559=CARTESIAN_POINT ( 'NONE',  ( -94.40760799030290684, -283.2289695933618532, -221.3595619813672783 ) ) ;
#14560=CARTESIAN_POINT ( 'NONE',  ( -79.19913533188103827, -280.4129184538163599, -210.2664962121950794 ) ) ;
#14561=CARTESIAN_POINT ( 'NONE',  ( 35.72838499098572385, -289.7788260859461502, -288.0448388335037748 ) ) ;
#14564=CARTESIAN_POINT ( 'NONE',  ( 10.30950500425925576, -296.3211470108273602, -329.0687937420232174 ) ) ;
#14566=CARTESIAN_POINT ( 'NONE',  ( -59.81798225130545887, -275.3431944377480249, -341.9140172150532635 ) ) ;
#14567=CARTESIAN_POINT ( 'NONE',  ( -108.6524110473766598, -289.3853857308030229, -298.9782689285400465 ) ) ;
#14568=CARTESIAN_POINT ( 'NONE',  ( -58.65857752850371298, -293.7323332621447776, -341.0154253634128168 ) ) ;
#14569=CARTESIAN_POINT ( 'NONE',  ( -105.9688156012415590, -277.5875196206615101, -243.9210882132089182 ) ) ;
#14570=CARTESIAN_POINT ( 'NONE',  ( 9.937728193903602403, -296.7896868835665600, -196.1410897974839713 ) ) ;
#14571=CARTESIAN_POINT ( 'NONE',  ( -52.48764953243479425, -293.1694022785607672, -198.3933322377198181 ) ) ;
#14572=CARTESIAN_POINT ( 'NONE',  ( -106.6379572354042153, -286.6233781216988064, -303.7686719486574134 ) ) ;
#14573=CARTESIAN_POINT ( 'NONE',  ( -47.55807765510908780, -293.6596596604184697, -345.9807806486943491 ) ) ;
#14574=CARTESIAN_POINT ( 'NONE',  ( -89.20899527712366250, -291.3971638969904916, -322.8608713941123369 ) ) ;
#14575=CARTESIAN_POINT ( 'NONE',  ( -98.23076809806080689, -288.1789549828755526, -315.8413649475575653 ) ) ;
#14577=CARTESIAN_POINT ( 'NONE',  ( 28.76497199245203618, -289.4118459033713293, -302.6919518190782696 ) ) ;
#14578=CARTESIAN_POINT ( 'NONE',  ( -95.89141555491156055, -290.7402959891028331, -314.2515159380465661 ) ) ;
#14580=CARTESIAN_POINT ( 'NONE',  ( -26.18714110429508679, -290.1182313084445923, -346.1475582652686853 ) ) ;
#14581=CARTESIAN_POINT ( 'NONE',  ( -108.0538028949382294, -276.9103282117731055, -244.1682332639914250 ) ) ;
#14582=CARTESIAN_POINT ( 'NONE',  ( -72.50094124074007595, -279.9329412640670398, -201.8660201664554279 ) ) ;
#14583=CARTESIAN_POINT ( 'NONE',  ( 22.50414704806151178, -281.8684927939851832, -318.7990479371065931 ) ) ;
#14584=CARTESIAN_POINT ( 'NONE',  ( 34.59533163545942358, -285.2782388284990702, -249.1010454784302510 ) ) ;
#14586=CARTESIAN_POINT ( 'NONE',  ( 32.23617289961259758, -279.3505710967674531, -244.3333083263952688 ) ) ;
#14587=CARTESIAN_POINT ( 'NONE',  ( -111.1728559817797333, -282.3789735861350323, -283.8362288018965387 ) ) ;
#14588=CARTESIAN_POINT ( 'NONE',  ( 201.7602898350666294, 289.7935801615433320, -82.39453394557040156 ) ) ;
#14589=CARTESIAN_POINT ( 'NONE',  ( -113.6837404213119811, -277.0526210999673253, -268.7295763606512651 ) ) ;
#14590=CARTESIAN_POINT ( 'NONE',  ( -110.3953052805852764, -283.1774024616702263, -293.7424718663654630 ) ) ;
#14591=CARTESIAN_POINT ( 'NONE',  ( -102.1782790309612921, -273.8165335113363881, -236.3571181942858743 ) ) ;
#14592=CARTESIAN_POINT ( 'NONE',  ( -110.4958876469581242, -292.2843612492586090, -260.2393685241858066 ) ) ;
#14593=CARTESIAN_POINT ( 'NONE',  ( -41.18146184613213734, -275.4301161149136874, -193.9950234166425957 ) ) ;
#14594=CARTESIAN_POINT ( 'NONE',  ( 33.60606453054442966, -275.4473897365221546, -287.6909929420282879 ) ) ;
#14595=CARTESIAN_POINT ( 'NONE',  ( -39.72783100643441401, -297.0822525087519921, -345.3359265764544830 ) ) ;
#14596=CARTESIAN_POINT ( 'NONE',  ( -12.22172293336124405, -288.9009801473249013, -343.2042606928760620 ) ) ;
#14597=CARTESIAN_POINT ( 'NONE',  ( 32.99314433328827789, -279.2736798469460382, -242.6079808221576570 ) ) ;
#14598=CARTESIAN_POINT ( 'NONE',  ( 4.143321927639485480, -292.4276496689330997, -205.4288719333016218 ) ) ;
#14599=CARTESIAN_POINT ( 'NONE',  ( -106.7906319551526337, -289.9186093409297769, -247.1177465376811426 ) ) ;
#14600=CARTESIAN_POINT ( 'NONE',  ( -73.66077835339257263, -293.5336571079670875, -336.0388376058859308 ) ) ;
#14603=CARTESIAN_POINT ( 'NONE',  ( -69.03863095940953087, -291.1313927356917475, -204.5195509894005852 ) ) ;
#14605=CARTESIAN_POINT ( 'NONE',  ( 32.49297727881272380, -288.0832418733486975, -238.3594161485135032 ) ) ;
#14606=CARTESIAN_POINT ( 'NONE',  ( 30.89617123739170168, -279.2666405000204009, -285.9686137636504668 ) ) ;
#14607=CARTESIAN_POINT ( 'NONE',  ( -16.58206775401803768, -293.8491766759644293, -344.3205625401920997 ) ) ;
#14608=CARTESIAN_POINT ( 'NONE',  ( -105.0038316043518449, -286.3326182936935993, -234.5386166278920257 ) ) ;
#14609=CARTESIAN_POINT ( 'NONE',  ( -108.3650178957309294, -284.6087072466704626, -253.4345796551743035 ) ) ;
#14611=CARTESIAN_POINT ( 'NONE',  ( 34.79610212069702868, -276.8746571627081039, -255.2382075643229769 ) ) ;
#14612=CARTESIAN_POINT ( 'NONE',  ( 37.26609728160536861, -291.5419346069503490, -268.0109338623844906 ) ) ;
#14613=CARTESIAN_POINT ( 'NONE',  ( 35.47616161325443329, -295.1389989878197184, -257.0418718988964883 ) ) ;
#14614=CARTESIAN_POINT ( 'NONE',  ( -3.699060005711096721, -275.3927422740687803, -335.5938035892796165 ) ) ;
#14617=CARTESIAN_POINT ( 'NONE',  ( 39.48073370224899747, -293.2899362352617345, -276.0418147363309345 ) ) ;
#14618=CARTESIAN_POINT ( 'NONE',  ( -0.2531660325689735203, -290.4753977054880920, -334.9631199203266192 ) ) ;
#14619=CARTESIAN_POINT ( 'NONE',  ( 202.4544974499246450, 295.8994530942177335, -54.00000000005819345 ) ) ;
#14620=CARTESIAN_POINT ( 'NONE',  ( -103.8922123153729729, -274.2536656754602973, -232.3199749452595597 ) ) ;
#14621=CARTESIAN_POINT ( 'NONE',  ( -62.60587658726665694, -286.3660555146923912, -201.7096536215012179 ) ) ;
#14622=ORIENTED_EDGE ( 'NONE', *, *, #32885, .F. ) ;
#14623=CARTESIAN_POINT ( 'NONE',  ( -98.38194974759099409, -278.2336065095286131, -223.7896486949875339 ) ) ;
#14624=CARTESIAN_POINT ( 'NONE',  ( 25.63594620929465506, -294.7880718475470303, -314.5103847847877887 ) ) ;
#14625=CARTESIAN_POINT ( 'NONE',  ( -59.68596496909783156, -287.4781480073875741, -342.7561406511053974 ) ) ;
#14626=CARTESIAN_POINT ( 'NONE',  ( -90.69436026410672014, -296.1167219692090953, -325.9253834831050654 ) ) ;
#14627=CARTESIAN_POINT ( 'NONE',  ( 2.248400320746489989, -292.9314914033633386, -208.9439779899522023 ) ) ;
#14631=CARTESIAN_POINT ( 'NONE',  ( 7.124056261922285138, -288.1654102198533565, -208.2839207440228790 ) ) ;
#14632=CARTESIAN_POINT ( 'NONE',  ( -19.11405058567864046, -292.3380690714489560, -350.3683826091709648 ) ) ;
#14634=CARTESIAN_POINT ( 'NONE',  ( -90.98111492513071141, -278.6635134398146079, -215.1858400577562520 ) ) ;
#14635=CARTESIAN_POINT ( 'NONE',  ( -20.96274796952394937, -284.8417872618542219, -343.4333311103478081 ) ) ;
#14636=CARTESIAN_POINT ( 'NONE',  ( -111.9536967999439412, -282.9191668208275132, -286.8431156798611141 ) ) ;
#14637=CARTESIAN_POINT ( 'NONE',  ( -64.36603136489249266, -287.4872895920181577, -339.7777504543332157 ) ) ;
#14638=CARTESIAN_POINT ( 'NONE',  ( 36.70365276891058670, -277.6173291475838028, -286.4714669451807936 ) ) ;
#14639=CARTESIAN_POINT ( 'NONE',  ( -55.31486126426177208, -298.3071144370772458, -199.4924226413671136 ) ) ;
#14642=CARTESIAN_POINT ( 'NONE',  ( 33.92016462287811152, -292.4725739042638111, -288.3330436326261292 ) ) ;
#14643=CARTESIAN_POINT ( 'NONE',  ( -107.9725817296657056, -278.7962843390746457, -251.8653763962713867 ) ) ;
#14644=CARTESIAN_POINT ( 'NONE',  ( -62.33601441295277823, -279.0669760907175601, -201.6114231959803931 ) ) ;
#14645=CARTESIAN_POINT ( 'NONE',  ( -52.49804125370265240, -274.9422038608369689, -195.1285865851194501 ) ) ;
#14646=CARTESIAN_POINT ( 'NONE',  ( -54.07724161490514803, -276.1823704047750994, -345.2581368141795224 ) ) ;
#14647=CARTESIAN_POINT ( 'NONE',  ( -64.53298115293586079, -181.9126970062073951, -359.6014539951557367 ) ) ;
#14649=CARTESIAN_POINT ( 'NONE',  ( -110.2322170070427632, -297.6866161885311044, -293.3303853515508308 ) ) ;
#14650=CARTESIAN_POINT ( 'NONE',  ( -110.4683760289727132, -275.2662352645559167, -253.7030783399848985 ) ) ;
#14653=CARTESIAN_POINT ( 'NONE',  ( 2.603983725294459095, -287.6814839605490306, -208.8910568579802316 ) ) ;
#14654=CARTESIAN_POINT ( 'NONE',  ( -91.20075834010039273, -287.0593250282994973, -216.7591043892576010 ) ) ;
#14655=CARTESIAN_POINT ( 'NONE',  ( 1.358523951712914846, -287.8686694867816982, -332.3787390613808270 ) ) ;
#14656=CARTESIAN_POINT ( 'NONE',  ( 34.52778608834048413, -281.4077939202252878, -297.8257107174369480 ) ) ;
#14657=VECTOR ( 'NONE', #16929, 999.9999999999998863 ) ;
#14658=CARTESIAN_POINT ( 'NONE',  ( -81.75323389522249329, -277.8361285208745244, -211.3558378910683757 ) ) ;
#14659=CARTESIAN_POINT ( 'NONE',  ( -98.38491818626364704, -286.9915617413628297, -228.0942186496788509 ) ) ;
#14660=CARTESIAN_POINT ( 'NONE',  ( -107.0947715153733242, -277.3468587693894847, -246.4302481829213320 ) ) ;
#14661=CARTESIAN_POINT ( 'NONE',  ( -98.04679154264975693, -279.2948238815476998, -311.7873820508854692 ) ) ;
#14662=CARTESIAN_POINT ( 'NONE',  ( 32.57710391074181189, -276.3254649268246794, -291.6023598868629279 ) ) ;
#14663=CARTESIAN_POINT ( 'NONE',  ( 19.32014905679930195, -287.0515246351829433, -321.9310498614780158 ) ) ;
#14664=CARTESIAN_POINT ( 'NONE',  ( -35.89196866455500867, -283.8372655698961466, -347.1990541950656848 ) ) ;
#14665=CARTESIAN_POINT ( 'NONE',  ( 39.64882686370275877, -282.0390317623076726, -269.9243541454740125 ) ) ;
#14669=CARTESIAN_POINT ( 'NONE',  ( -31.89159190179160319, -290.8446213608816038, -345.9813543484453362 ) ) ;
#14670=CARTESIAN_POINT ( 'NONE',  ( -110.7542129672360858, -289.5088822208843453, -248.8227514750625176 ) ) ;
#14671=CARTESIAN_POINT ( 'NONE',  ( -106.5247456105528840, -271.9293649090562326, -246.3379070041839043 ) ) ;
#14672=CARTESIAN_POINT ( 'NONE',  ( 29.39130356909437580, -292.4036454861914649, -232.1509229570749540 ) ) ;
#14673=CARTESIAN_POINT ( 'NONE',  ( -110.3121900072888337, -288.8962913654746103, -280.7481921873157944 ) ) ;
#14674=CARTESIAN_POINT ( 'NONE',  ( 29.66533389325711667, -291.3718119426521298, -238.8071165447032058 ) ) ;
#14675=CARTESIAN_POINT ( 'NONE',  ( 8.238464385818897284, -289.6174307781887478, -327.8900594511158602 ) ) ;
#14676=CARTESIAN_POINT ( 'NONE',  ( -20.19161114001083490, -291.3376638359845856, -345.3538533559490702 ) ) ;
#14677=CARTESIAN_POINT ( 'NONE',  ( 13.27326456308053970, -290.3449888223296398, -325.7770311679109909 ) ) ;
#14678=CARTESIAN_POINT ( 'NONE',  ( -44.69180684110243362, -289.9593064400704634, -195.5030100218429254 ) ) ;
#14679=CARTESIAN_POINT ( 'NONE',  ( -112.0355377871429567, -292.6462531215783542, -263.0450503807348355 ) ) ;
#14680=CARTESIAN_POINT ( 'NONE',  ( -110.1051012436151808, -285.3785214281243725, -279.0982878643101230 ) ) ;
#14681=CARTESIAN_POINT ( 'NONE',  ( 0.7485623503338053597, -294.5586054161193488, -205.5007167355416300 ) ) ;
#14684=CARTESIAN_POINT ( 'NONE',  ( 6.911740759338740325, -300.5221789476098024, -194.7867625352656091 ) ) ;
#14685=CARTESIAN_POINT ( 'NONE',  ( 34.86127483211399181, -280.9046857088136449, -282.1650213229119117 ) ) ;
#14686=CARTESIAN_POINT ( 'NONE',  ( -105.9529299669932669, -282.1552425056159450, -300.6513769083413763 ) ) ;
#14687=CARTESIAN_POINT ( 'NONE',  ( -94.53822927535699705, -295.0515271794511136, -321.6907221965095687 ) ) ;
#14688=CARTESIAN_POINT ( 'NONE',  ( 21.50061224621594747, -273.1690913463195329, -225.4453017140346844 ) ) ;
#14689=CARTESIAN_POINT ( 'NONE',  ( -110.0071900377795231, -276.8416971055762019, -254.1460980003063526 ) ) ;
#14690=CARTESIAN_POINT ( 'NONE',  ( -86.44211597670678771, -298.6682237016093495, -215.6766353540418208 ) ) ;
#14691=CARTESIAN_POINT ( 'NONE',  ( -31.28850420442002545, -272.7018945833042380, -194.1773066328008213 ) ) ;
#14692=CARTESIAN_POINT ( 'NONE',  ( 34.79048186211772986, -294.7867466033989672, -255.7898023258425724 ) ) ;
#14694=CARTESIAN_POINT ( 'NONE',  ( 16.28444113704671281, -295.0687007466637510, -320.1289660382206534 ) ) ;
#14696=CARTESIAN_POINT ( 'NONE',  ( -26.82516625758425732, -284.2052313124946750, -195.6910057279293369 ) ) ;
#14697=CARTESIAN_POINT ( 'NONE',  ( -102.5323343252196366, -296.9993750490144748, -237.3976725173052387 ) ) ;
#14698=CARTESIAN_POINT ( 'NONE',  ( -114.3266410319141357, -284.5927567678380115, -267.1144071126789754 ) ) ;
#14699=CARTESIAN_POINT ( 'NONE',  ( 25.53028977124331078, -286.6306813682153347, -225.9215329488652912 ) ) ;
#14700=CARTESIAN_POINT ( 'NONE',  ( 7.801986856872882292, -290.6701741160864003, -210.6779884661212634 ) ) ;
#14702=CARTESIAN_POINT ( 'NONE',  ( -42.40917472496116147, -279.1869394266634004, -193.6898748610606447 ) ) ;
#14704=CARTESIAN_POINT ( 'NONE',  ( -114.2704648735229114, -276.0523547857347353, -270.3284710469133074 ) ) ;
#14706=CARTESIAN_POINT ( 'NONE',  ( 34.90987780542751295, -286.5165429661380472, -283.2777735735420492 ) ) ;
#14707=CARTESIAN_POINT ( 'NONE',  ( -71.78003240611128888, -288.4169604927631099, -338.8847911248911373 ) ) ;
#14710=CARTESIAN_POINT ( 'NONE',  ( -102.1603456800654470, -297.6758759337017182, -305.6454431441087536 ) ) ;
#14711=CARTESIAN_POINT ( 'NONE',  ( -36.77529057724611050, -281.4844069552212886, -193.9394985469993742 ) ) ;
#14712=CARTESIAN_POINT ( 'NONE',  ( -103.7910480535068700, -295.0428250785489581, -234.7133177948825278 ) ) ;
#14713=CARTESIAN_POINT ( 'NONE',  ( 25.57509289597656021, -281.7289783874593923, -307.5226576701639942 ) ) ;
#14714=CARTESIAN_POINT ( 'NONE',  ( 15.48022856860141871, -294.4963516356596074, -326.3865037755567187 ) ) ;
#14715=CARTESIAN_POINT ( 'NONE',  ( 32.53720705406479397, -285.2582028480800886, -241.4797112760513471 ) ) ;
#14716=CARTESIAN_POINT ( 'NONE',  ( -53.35885485968260866, -281.8470233110237473, -197.0382460943236254 ) ) ;
#14717=CARTESIAN_POINT ( 'NONE',  ( -66.90336041185956617, -296.7137356709977780, -203.3435394562554279 ) ) ;
#14720=CARTESIAN_POINT ( 'NONE',  ( -7.821063966410090273, -284.6432783730629694, -338.9204269455259464 ) ) ;
#14721=LINE ( 'NONE', #28914, #50446 ) ;
#14722=CARTESIAN_POINT ( 'NONE',  ( -54.49178911615187104, -286.7666405000204009, -345.3538533559490702 ) ) ;
#14723=CARTESIAN_POINT ( 'NONE',  ( 39.46152690502968596, -274.7955078877226924, -274.0464369994128901 ) ) ;
#14724=CARTESIAN_POINT ( 'NONE',  ( -79.52897508416512551, -291.2980185364006047, -210.7237132508768127 ) ) ;
#14725=CARTESIAN_POINT ( 'NONE',  ( 22.38512852578466195, -283.6706928002748782, -313.5500070594430895 ) ) ;
#14726=CARTESIAN_POINT ( 'NONE',  ( 1.011003716962067145, -276.1734422399819096, -207.3094683400648535 ) ) ;
#14727=CARTESIAN_POINT ( 'NONE',  ( 23.62739151063188814, -283.7669727043859211, -316.0689978515228518 ) ) ;
#14728=CARTESIAN_POINT ( 'NONE',  ( 34.61694634458199005, -280.5376183216969821, -284.8840297448066394 ) ) ;
#14729=CARTESIAN_POINT ( 'NONE',  ( -92.41974689240720409, -279.8399450613550243, -321.3425179418276798 ) ) ;
#14730=CARTESIAN_POINT ( 'NONE',  ( -34.75943534448137484, -298.0836462427581637, -193.3611179409975591 ) ) ;
#14731=CARTESIAN_POINT ( 'NONE',  ( 28.50364904711516800, -274.8632677669531290, -230.3418931644260681 ) ) ;
#14732=CARTESIAN_POINT ( 'NONE',  ( 36.13136501124787969, -295.3165694703349118, -258.3223507771058394 ) ) ;
#14733=DIRECTION ( 'NONE',  ( 0.000000000000000000, 0.000000000000000000, 1.000000000000000000 ) ) ;
#14735=CARTESIAN_POINT ( 'NONE',  ( -36.31533462420337344, -293.1790403635137636, -346.1318633065986887 ) ) ;
#14736=CARTESIAN_POINT ( 'NONE',  ( -16.61720812348815812, -273.8347603314010144, -200.2477907273416804 ) ) ;
#14737=CARTESIAN_POINT ( 'NONE',  ( -4.916502636190464237, -293.9915233032718334, -201.2864169476227403 ) ) ;
#14738=CARTESIAN_POINT ( 'NONE',  ( -54.42813229853333468, -279.7662352645560304, -345.3683826091709648 ) ) ;
#14739=CARTESIAN_POINT ( 'NONE',  ( -42.04499282550026606, -293.1991759095635075, -193.9027125799210012 ) ) ;
#14740=CARTESIAN_POINT ( 'NONE',  ( -73.21590917287862510, -291.5291735430358244, -336.0350820297179553 ) ) ;
#14741=CARTESIAN_POINT ( 'NONE',  ( -92.33193978249501299, -275.8402696384227966, -321.1918373651718639 ) ) ;
#14742=CARTESIAN_POINT ( 'NONE',  ( -6.896772956942379906, -278.5695899812970424, -338.2906447746437948 ) ) ;
#14743=CARTESIAN_POINT ( 'NONE',  ( 13.31729013591951549, -292.4172663218649291, -324.9751306684927386 ) ) ;
#14744=CARTESIAN_POINT ( 'NONE',  ( 36.12758844938015557, -283.1772059113966407, -251.8524951396767335 ) ) ;
#14746=CARTESIAN_POINT ( 'NONE',  ( 15.83834964011666990, -281.9397405518457163, -320.4737450861345565 ) ) ;
#14747=CARTESIAN_POINT ( 'NONE',  ( -7.669334412943259238, -281.5117166814559937, -199.6288191039427602 ) ) ;
#14748=CARTESIAN_POINT ( 'NONE',  ( -93.15281200929155148, -282.6270664633530032, -322.8506155782857263 ) ) ;
#14749=CARTESIAN_POINT ( 'NONE',  ( -104.7631951829051076, -279.0169628438342215, -307.0648264724873115 ) ) ;
#14751=CARTESIAN_POINT ( 'NONE',  ( 35.06585357261640468, -276.7644866612782266, -246.1145303415782735 ) ) ;
#14752=CARTESIAN_POINT ( 'NONE',  ( -37.37352853689063181, -288.5519495502701375, -200.3611179825600459 ) ) ;
#14754=CARTESIAN_POINT ( 'NONE',  ( -42.01780419505228537, -299.9933605374345689, -195.5070285774019112 ) ) ;
#14756=CARTESIAN_POINT ( 'NONE',  ( -111.8112106427697228, -276.4971519770018062, -276.1826063638703204 ) ) ;
#14757=CARTESIAN_POINT ( 'NONE',  ( -79.05709251131023052, -293.2584519606065214, -206.7860050813560235 ) ) ;
#14758=CARTESIAN_POINT ( 'NONE',  ( 16.81927857615029964, -292.1975518639670781, -221.1902152464070639 ) ) ;
#14759=CARTESIAN_POINT ( 'NONE',  ( -113.1103257176929446, -290.2270975042544592, -256.9954051471577259 ) ) ;
#14761=CARTESIAN_POINT ( 'NONE',  ( -1.002512906155358596, -293.1542530978201171, -337.5924762793551963 ) ) ;
#14762=CARTESIAN_POINT ( 'NONE',  ( -100.2810557584299715, -283.4784496777049299, -231.7270852882678867 ) ) ;
#14763=CARTESIAN_POINT ( 'NONE',  ( -84.63385005270421857, -293.2528883724849038, -213.1394609550296479 ) ) ;
#14764=CARTESIAN_POINT ( 'NONE',  ( -44.06857364976190183, -284.4454302669668664, -196.9754455050674267 ) ) ;
#14765=CARTESIAN_POINT ( 'NONE',  ( -13.35267622803792165, -284.0493021278487049, -339.8828531023201549 ) ) ;
#14766=CARTESIAN_POINT ( 'NONE',  ( -69.24853949100405259, -290.4029732288698256, -340.1950767248400780 ) ) ;
#14767=CARTESIAN_POINT ( 'NONE',  ( -3.125819734950805895, -281.0093317473082948, -205.7925953410922091 ) ) ;
#14768=CARTESIAN_POINT ( 'NONE',  ( 37.67619781785987243, -292.1513893729710389, -254.7943891658774760 ) ) ;
#14769=CARTESIAN_POINT ( 'NONE',  ( -41.74107220276406593, -289.9090497843407093, -347.0867908904371006 ) ) ;
#14770=CARTESIAN_POINT ( 'NONE',  ( 39.03027521805085343, -288.1665080889038677, -280.1091622905239547 ) ) ;
#14771=CARTESIAN_POINT ( 'NONE',  ( -67.54963498449838255, -285.8111233478732061, -203.9045105139182965 ) ) ;
#14774=CARTESIAN_POINT ( 'NONE',  ( 38.37337241005804600, -295.4474545257387490, -273.1057980142564361 ) ) ;
#14775=CARTESIAN_POINT ( 'NONE',  ( -64.10943491397799221, -294.0790027931365671, -342.0324975348340786 ) ) ;
#14776=CARTESIAN_POINT ( 'NONE',  ( -102.3592740409991961, -278.0691540720724788, -236.5443515814337729 ) ) ;
#14777=CARTESIAN_POINT ( 'NONE',  ( -114.2799287340801158, -272.0957458231548571, -267.4896894357692076 ) ) ;
#14778=CARTESIAN_POINT ( 'NONE',  ( -66.34365821927771378, -293.9188012278380597, -338.1076616619154720 ) ) ;
#14779=CARTESIAN_POINT ( 'NONE',  ( 19.09544620236716028, -277.9837771567024447, -318.2445444438492359 ) ) ;
#14780=CARTESIAN_POINT ( 'NONE',  ( -109.7342660377521497, -270.9049628485799985, -253.9239076013647320 ) ) ;
#14781=CARTESIAN_POINT ( 'NONE',  ( 18.77028751652482441, -294.0886343375929073, -223.0475327406124393 ) ) ;
#14782=CARTESIAN_POINT ( 'NONE',  ( -100.4254895946988455, -297.1196362108358358, -307.8062092200646589 ) ) ;
#14784=CARTESIAN_POINT ( 'NONE',  ( -112.2906034502529167, -294.6334884781005599, -263.9996424628623117 ) ) ;
#14785=CARTESIAN_POINT ( 'NONE',  ( -70.69234694344012837, -298.2751821990243570, -201.0715289794235900 ) ) ;
#14786=CARTESIAN_POINT ( 'NONE',  ( -84.46649122563921708, -275.4034827066340085, -212.0151266066184235 ) ) ;
#14787=CARTESIAN_POINT ( 'NONE',  ( -106.2499222435548489, -291.1641629305350989, -295.1616295242016577 ) ) ;
#14788=CARTESIAN_POINT ( 'NONE',  ( -82.36951343899568201, -296.0193558748632086, -327.9110894352050991 ) ) ;
#14789=CARTESIAN_POINT ( 'NONE',  ( -112.4078610844074717, -280.6236121945696596, -263.1959479991191415 ) ) ;
#14790=CARTESIAN_POINT ( 'NONE',  ( -111.6031672020957473, -277.4692574168315673, -251.9081571855818993 ) ) ;
#14791=CARTESIAN_POINT ( 'NONE',  ( 9.140588080326475406, -281.7810914984025885, -331.6204819131916679 ) ) ;
#14792=CARTESIAN_POINT ( 'NONE',  ( 18.82308612344793985, -275.6180919769613524, -322.8856795886061946 ) ) ;
#14793=CARTESIAN_POINT ( 'NONE',  ( -72.10256061430081331, -281.5954978469592902, -336.1866204754747400 ) ) ;
#14794=CARTESIAN_POINT ( 'NONE',  ( -47.98665536977560464, -278.3189190905283681, -194.8550325238680330 ) ) ;
#14795=CARTESIAN_POINT ( 'NONE',  ( 7.474386834444151972, -278.6611978139957273, -209.9511716035584072 ) ) ;
#14796=CARTESIAN_POINT ( 'NONE',  ( -97.27526463676956325, -295.8269545473135054, -227.8262931449855273 ) ) ;
#14797=CARTESIAN_POINT ( 'NONE',  ( 20.43589238840171873, -278.2124272923527997, -318.2007428124951502 ) ) ;
#14799=CARTESIAN_POINT ( 'NONE',  ( 33.90591496058647181, -291.2543755690602438, -245.6635697208846523 ) ) ;
#14800=CARTESIAN_POINT ( 'NONE',  ( -113.1333019889379443, -290.3812843703086060, -284.0235685012721092 ) ) ;
#14801=CARTESIAN_POINT ( 'NONE',  ( 23.81996640873066085, -276.9591021996823201, -226.6438118749740624 ) ) ;
#14802=CARTESIAN_POINT ( 'NONE',  ( -91.35184219392029092, -295.2819183494752906, -218.4899523001131172 ) ) ;
#14804=CARTESIAN_POINT ( 'NONE',  ( -113.4409205647635446, -283.6113440162257575, -281.3706060883149007 ) ) ;
#14806=CARTESIAN_POINT ( 'NONE',  ( -96.61789992795272042, -281.9218930005891934, -316.3308250677001183 ) ) ;
#14808=CARTESIAN_POINT ( 'NONE',  ( 4.743815059678500035, -291.4292168696130716, -210.1661205989241807 ) ) ;
#14809=CARTESIAN_POINT ( 'NONE',  ( -107.6954548529433708, -283.0030790125842373, -246.5103426102602384 ) ) ;
#14812=CARTESIAN_POINT ( 'NONE',  ( -30.60257476703284496, -290.1372171987408706, -195.6644993311574581 ) ) ;
#14813=CARTESIAN_POINT ( 'NONE',  ( -65.01892186425033060, -281.8871162181939098, -341.4855263138263126 ) ) ;
#14814=CARTESIAN_POINT ( 'NONE',  ( -83.49132363877386354, -279.2968838335467012, -328.0172618089705452 ) ) ;
#14815=CARTESIAN_POINT ( 'NONE',  ( -111.9763485445742077, -285.9741187170923240, -253.1077711664929666 ) ) ;
#14816=CARTESIAN_POINT ( 'NONE',  ( -71.17822123322197569, -285.5923384798751954, -205.6765770202761701 ) ) ;
#14817=CARTESIAN_POINT ( 'NONE',  ( -102.3691914221685693, -279.5119057565265734, -304.8110859297080992 ) ) ;
#14818=CARTESIAN_POINT ( 'NONE',  ( -108.6413301881170526, -279.1383884904341812, -286.8167415670671971 ) ) ;
#14819=CARTESIAN_POINT ( 'NONE',  ( -109.5586269592996871, -286.2919024084290527, -290.6025638230204891 ) ) ;
#14822=CARTESIAN_POINT ( 'NONE',  ( -113.6014641939272281, -296.5198734781723715, -259.6145429405056007 ) ) ;
#14823=CARTESIAN_POINT ( 'NONE',  ( 23.31260991251044246, -290.1268068552267891, -313.8686055902316525 ) ) ;
#14825=CARTESIAN_POINT ( 'NONE',  ( 36.60358173371528068, -278.4805209788416391, -305.9350535429201159 ) ) ;
#14826=ORIENTED_EDGE ( 'NONE', *, *, #63185, .T. ) ;
#14827=CARTESIAN_POINT ( 'NONE',  ( 22.49270005178255616, -291.3141389837169868, -223.1567353524231407 ) ) ;
#14828=CARTESIAN_POINT ( 'NONE',  ( 25.53227725579910157, -288.5476298815528935, -231.9219358955942596 ) ) ;
#14829=CARTESIAN_POINT ( 'NONE',  ( -109.2798108946321918, -280.5387685725110600, -252.9576058188420689 ) ) ;
#14830=CARTESIAN_POINT ( 'NONE',  ( 37.25370945427000891, -289.1868351347378621, -286.9778211760788054 ) ) ;
#14831=CARTESIAN_POINT ( 'NONE',  ( -3.265240683244684305, -289.9268033375313962, -338.8745095060730250 ) ) ;
#14832=CARTESIAN_POINT ( 'NONE',  ( -79.47984415947874481, -285.6214919268298900, -332.4044694729619778 ) ) ;
#14833=CARTESIAN_POINT ( 'NONE',  ( -110.5503471914902747, -279.0209539291169563, -246.3278015985067384 ) ) ;
#14835=CARTESIAN_POINT ( 'NONE',  ( -22.40654436401687732, -292.9421965613617544, -344.4303782564640528 ) ) ;
#14836=CARTESIAN_POINT ( 'NONE',  ( 17.22461029268343324, -280.6376626442193469, -215.9584780100617536 ) ) ;
#14837=CARTESIAN_POINT ( 'NONE',  ( -63.76821030538676638, -275.5643605123421480, -200.9751732569491480 ) ) ;
#14839=CARTESIAN_POINT ( 'NONE',  ( -95.99890600148557951, -293.6948066931273615, -223.6242672951989618 ) ) ;
#14840=CARTESIAN_POINT ( 'NONE',  ( -52.32360105921783600, -272.1028482312019037, -195.8123186308396555 ) ) ;
#14842=CARTESIAN_POINT ( 'NONE',  ( -102.2076343630536712, -278.5179866330135496, -236.6296216210916157 ) ) ;
#14843=CARTESIAN_POINT ( 'NONE',  ( 39.15681735701561195, -276.6954857365176963, -265.4498619058410895 ) ) ;
#14844=CARTESIAN_POINT ( 'NONE',  ( -97.37384333853346163, -298.5669582364377561, -227.7992019136804345 ) ) ;
#14845=CARTESIAN_POINT ( 'NONE',  ( -113.9742949977663642, -283.5440592715557386, -275.6894695110132716 ) ) ;
#14846=CARTESIAN_POINT ( 'NONE',  ( -87.39844968253277102, -291.5215233255315184, -324.9493900710586445 ) ) ;
#14847=CARTESIAN_POINT ( 'NONE',  ( -34.10323442049305243, -299.6121161593194415, -194.0536266358848820 ) ) ;
#14848=CARTESIAN_POINT ( 'NONE',  ( -40.43964752190774448, -299.2192245205288259, -193.7690007450092935 ) ) ;
#14849=CARTESIAN_POINT ( 'NONE',  ( -45.26002190593178653, -297.1527124863017661, -344.8260905709048529 ) ) ;
#14850=CARTESIAN_POINT ( 'NONE',  ( -66.04179726966926012, -281.4284039956132801, -339.4860786965474517 ) ) ;
#14851=CARTESIAN_POINT ( 'NONE',  ( -77.15469256056981351, -291.2009771039146244, -204.4158835851181379 ) ) ;
#14852=CARTESIAN_POINT ( 'NONE',  ( -91.37011123717476835, -271.2988866390000453, -218.8373026335324312 ) ) ;
#14853=CARTESIAN_POINT ( 'NONE',  ( -30.97125657269966226, -287.7314797219319189, -194.4147152786025003 ) ) ;
#14854=CARTESIAN_POINT ( 'NONE',  ( -94.35331839890713468, -288.8234033255558302, -316.4469233550374270 ) ) ;
#14855=CARTESIAN_POINT ( 'NONE',  ( -20.78800910493833953, -109.0397813191330840, -362.5271799116017064 ) ) ;
#14857=CARTESIAN_POINT ( 'NONE',  ( -110.9790243079734466, -288.8693395513073483, -290.7608920363040284 ) ) ;
#14858=CARTESIAN_POINT ( 'NONE',  ( -84.70196802366683642, -289.3924907514538631, -326.0074665535559575 ) ) ;
#14860=CARTESIAN_POINT ( 'NONE',  ( -35.17081953721390875, -287.1584438759344380, -193.6878694151492937 ) ) ;
#14861=CARTESIAN_POINT ( 'NONE',  ( -19.00753910479205544, -277.1428452809773262, -341.0431243650499482 ) ) ;
#14862=CARTESIAN_POINT ( 'NONE',  ( 37.76506609359885402, -292.6672036442209901, -285.8680899183771658 ) ) ;
#14863=CARTESIAN_POINT ( 'NONE',  ( -70.41874318633490759, -284.1281262113888033, -339.7961764470020967 ) ) ;
#14864=CARTESIAN_POINT ( 'NONE',  ( 24.55632322577920590, -283.6695539827626362, -315.0077657658079602 ) ) ;
#14865=CARTESIAN_POINT ( 'NONE',  ( -47.24943568301077335, -283.5080511325226666, -346.6997128585537666 ) ) ;
#14866=CARTESIAN_POINT ( 'NONE',  ( -6.764438461699285199, -280.7982115897678455, -204.0366961401643948 ) ) ;
#14867=CARTESIAN_POINT ( 'NONE',  ( -113.6816706259712220, -273.8610821628187750, -284.1793481324285722 ) ) ;
#14868=CARTESIAN_POINT ( 'NONE',  ( 198.6360497827117513, 289.4354249690432539, -97.31417216244363999 ) ) ;
#14869=CARTESIAN_POINT ( 'NONE',  ( -112.7803442879496032, -270.5759482646675451, -270.3359561730730434 ) ) ;
#14870=CARTESIAN_POINT ( 'NONE',  ( -93.89669983061651237, -272.4055451961618246, -223.9288858873298977 ) ) ;
#14871=CARTESIAN_POINT ( 'NONE',  ( -39.11271196219436064, -294.5814751962054743, -347.2791940151172412 ) ) ;
#14872=CARTESIAN_POINT ( 'NONE',  ( 122.2538704333025805, 147.2434944315820644, -260.5076579305660402 ) ) ;
#14873=CARTESIAN_POINT ( 'NONE',  ( -87.69910126009085616, -272.0511269554788214, -212.6935573124585801 ) ) ;
#14874=CARTESIAN_POINT ( 'NONE',  ( -111.0275985750256069, -298.2903148450803883, -279.7857737810234084 ) ) ;
#14875=CARTESIAN_POINT ( 'NONE',  ( 34.47436211061453548, -288.6627780919735073, -254.7503305551154256 ) ) ;
#14877=CARTESIAN_POINT ( 'NONE',  ( -8.465390047287353781, -295.6246563919564778, -341.5439308367457443 ) ) ;
#14878=CARTESIAN_POINT ( 'NONE',  ( -2.162255260902521847, -287.0231850229944826, -206.2700285039655910 ) ) ;
#14879=CARTESIAN_POINT ( 'NONE',  ( -83.38349125174104870, -272.3583117319657276, -208.9624029320040961 ) ) ;
#14880=CARTESIAN_POINT ( 'NONE',  ( -24.92381222732600676, -295.7005895693181401, -346.2435282884025582 ) ) ;
#14881=CARTESIAN_POINT ( 'NONE',  ( 19.48846531651184577, -294.7508599749521636, -322.3025787969735916 ) ) ;
#14882=CARTESIAN_POINT ( 'NONE',  ( -52.37184258195792097, -292.0210930969362266, -198.8732677104928541 ) ) ;
#14884=CARTESIAN_POINT ( 'NONE',  ( -102.9907636591982794, -274.9686288757571901, -232.8459701381500224 ) ) ;
#14885=CARTESIAN_POINT ( 'NONE',  ( 19.75024487983085564, -273.6501420795791546, -219.2094889890695413 ) ) ;
#14887=CARTESIAN_POINT ( 'NONE',  ( -84.52424538857647462, -278.9300216042117881, -209.5208926071358064 ) ) ;
#14888=CARTESIAN_POINT ( 'NONE',  ( 5.659244314338219617, -273.0450854044192965, -210.3199547955777007 ) ) ;
#14889=CARTESIAN_POINT ( 'NONE',  ( -62.14716549262230672, -274.8015128918820551, -201.3762286118088412 ) ) ;
#14890=CARTESIAN_POINT ( 'NONE',  ( 23.98400156855259269, -275.9404525566801567, -230.3290463462648745 ) ) ;
#14891=CARTESIAN_POINT ( 'NONE',  ( -29.18694711724390345, -299.7527560072383039, -194.1589351109550705 ) ) ;
#14892=CARTESIAN_POINT ( 'NONE',  ( 18.63805300244820273, -274.2721810933783217, -320.8251831716453921 ) ) ;
#14893=CARTESIAN_POINT ( 'NONE',  ( -77.99955609782713850, -296.2656886075365037, -331.1744680234588714 ) ) ;
#14894=CARTESIAN_POINT ( 'NONE',  ( -37.01098419482438828, -293.6226248903224132, -343.9621299455653798 ) ) ;
#14895=CARTESIAN_POINT ( 'NONE',  ( -109.6767582881953729, -278.7113859919203378, -296.7307906927459840 ) ) ;
#14896=CARTESIAN_POINT ( 'NONE',  ( 30.17400937081869827, -275.3451828110256088, -242.4681892881451688 ) ) ;
#14897=CARTESIAN_POINT ( 'NONE',  ( -107.4673622681433471, -283.6309704386822546, -239.6396735085565695 ) ) ;
#14898=CARTESIAN_POINT ( 'NONE',  ( -106.6739170244196373, -298.1724354942691093, -299.5314257026497557 ) ) ;
#14900=CARTESIAN_POINT ( 'NONE',  ( -87.79849167931553211, -284.5219912584266240, -217.3826892305910974 ) ) ;
#14901=EDGE_CURVE ( 'NONE', #89916, #85520, #53589, .T. ) ;
#14902=CARTESIAN_POINT ( 'NONE',  ( -94.40138141946381722, -276.1327314016297123, -317.5208471865127535 ) ) ;
#14903=CARTESIAN_POINT ( 'NONE',  ( -36.47731876809259433, -275.6158716797094144, -343.9578404526012037 ) ) ;
#14904=CARTESIAN_POINT ( 'NONE',  ( -71.18510159373920487, -285.4989856455753738, -337.3051577066497657 ) ) ;
#14905=CARTESIAN_POINT ( 'NONE',  ( -76.55506268344306875, -278.7943052725789812, -332.4647621242654054 ) ) ;
#14907=CARTESIAN_POINT ( 'NONE',  ( 28.39540212061361757, -274.4589258740609807, -308.8977732851108726 ) ) ;
#14908=CARTESIAN_POINT ( 'NONE',  ( -67.94987770663411197, -281.6514772247853102, -201.6945566625774404 ) ) ;
#14911=CARTESIAN_POINT ( 'NONE',  ( 22.16874578847162169, -290.1066633111701094, -316.9418243979674799 ) ) ;
#14912=CARTESIAN_POINT ( 'NONE',  ( -20.75435260425014761, -290.2647829228209275, -197.1657367044340674 ) ) ;
#14913=CARTESIAN_POINT ( 'NONE',  ( 82.16406924513974275, -298.3597564528348016, -196.9763042694495994 ) ) ;
#14914=CARTESIAN_POINT ( 'NONE',  ( -103.6428112044271614, -271.6629357506310498, -238.6529779140942651 ) ) ;
#14915=CARTESIAN_POINT ( 'NONE',  ( -80.22525522428877309, -289.6045552778905403, -209.7021980574301949 ) ) ;
#14916=CARTESIAN_POINT ( 'NONE',  ( 201.9366853066881333, 285.6703355482916322, -112.9373754057687478 ) ) ;
#14917=CARTESIAN_POINT ( 'NONE',  ( 98.97854452771385070, -297.7583178930348708, -195.4075969279095091 ) ) ;
#14918=CARTESIAN_POINT ( 'NONE',  ( -72.86839492463008128, -287.9939380051652051, -337.9076741874630443 ) ) ;
#14919=CARTESIAN_POINT ( 'NONE',  ( -37.52223829737051375, -284.6546140882725240, -344.1734651764551245 ) ) ;
#14920=CARTESIAN_POINT ( 'NONE',  ( -84.86152418970716838, -283.6468349526077191, -211.0665960397071501 ) ) ;
#14922=CARTESIAN_POINT ( 'NONE',  ( -21.24176701983879312, -284.2669915878626625, -342.2200088793306350 ) ) ;
#14923=CARTESIAN_POINT ( 'NONE',  ( -109.0893247005254665, -285.5433910475724133, -256.0474847739077404 ) ) ;
#14924=CARTESIAN_POINT ( 'NONE',  ( -111.2497337784899827, -292.3433849835209912, -285.1236716151495330 ) ) ;
#14925=CARTESIAN_POINT ( 'NONE',  ( -10.35900340810864684, -274.7279552595405789, -198.2094853670780310 ) ) ;
#14926=CARTESIAN_POINT ( 'NONE',  ( -112.7491741434206602, -288.6931543503907847, -265.5624662647101104 ) ) ;
#14927=CARTESIAN_POINT ( 'NONE',  ( 3.501501106008682029, -276.5194132478321194, -335.6989378172016245 ) ) ;
#14928=CARTESIAN_POINT ( 'NONE',  ( 17.38175315535427146, -296.2455703932877782, -321.1271545024767420 ) ) ;
#14930=CARTESIAN_POINT ( 'NONE',  ( -85.28047601435908120, -292.1948066931273615, -330.5268031993605859 ) ) ;
#14931=CARTESIAN_POINT ( 'NONE',  ( 1.346770494103801230, -281.2087452807162435, -332.9060995216835863 ) ) ;
#14932=CARTESIAN_POINT ( 'NONE',  ( -111.1901092267232798, -276.7324355051349585, -256.2766651246321317 ) ) ;
#14933=CARTESIAN_POINT ( 'NONE',  ( -63.30285051703177146, -272.1998341367411740, -198.6064914934049739 ) ) ;
#14934=CARTESIAN_POINT ( 'NONE',  ( 34.94369633539486841, -274.7560950019083634, -259.3812303385336122 ) ) ;
#14935=CARTESIAN_POINT ( 'NONE',  ( 22.35509582956093055, -294.4732058097428649, -227.1308678496267248 ) ) ;
#14936=CARTESIAN_POINT ( 'NONE',  ( 34.00737184365192434, -294.7112127627005407, -286.9305922991796933 ) ) ;
#14937=CARTESIAN_POINT ( 'NONE',  ( 37.48119411981927840, -294.7813119015780217, -254.8005848664153916 ) ) ;
#14938=CARTESIAN_POINT ( 'NONE',  ( 6.346222210225488602, -295.7879424278364127, -333.2322374880150733 ) ) ;
#14939=CARTESIAN_POINT ( 'NONE',  ( -53.15144538113155193, -295.0937319614895387, -341.6805706454919118 ) ) ;
#14940=CARTESIAN_POINT ( 'NONE',  ( -98.97842001112121579, -291.9725364729412149, -313.1144018941114382 ) ) ;
#14941=CARTESIAN_POINT ( 'NONE',  ( -37.31212119221935808, -283.2184342017803260, -347.3741776089751738 ) ) ;
#14942=CARTESIAN_POINT ( 'NONE',  ( -87.20533637919137959, -271.5059727849838964, -213.2482149604902304 ) ) ;
#14943=CARTESIAN_POINT ( 'NONE',  ( 20.28816140619682784, -286.6930171452784748, -219.2157929538252858 ) ) ;
#14944=CARTESIAN_POINT ( 'NONE',  ( -54.30372325327672911, -279.2508434928289489, -343.1064964808805939 ) ) ;
#14945=CARTESIAN_POINT ( 'NONE',  ( -79.52501797105988146, -284.2633591061516540, -210.2346145330780871 ) ) ;
#14947=CARTESIAN_POINT ( 'NONE',  ( -74.69040791796525980, -287.5491056504151857, -335.4001422358676905 ) ) ;
#14948=CARTESIAN_POINT ( 'NONE',  ( -100.8428064840771583, -277.2444587217430580, -228.9393001400984247 ) ) ;
#14949=CARTESIAN_POINT ( 'NONE',  ( 121.1498776811041438, 150.0802918209077177, -263.8330885344481658 ) ) ;
#14950=CARTESIAN_POINT ( 'NONE',  ( 19.82209492063704204, -282.0620784621206667, -219.3481717810390137 ) ) ;
#14951=CARTESIAN_POINT ( 'NONE',  ( -104.9544096972042553, -289.1394976908217131, -306.7113823151653378 ) ) ;
#14952=CARTESIAN_POINT ( 'NONE',  ( -102.9069449596131562, -279.6399374951424193, -309.2928741573435900 ) ) ;
#14953=CARTESIAN_POINT ( 'NONE',  ( -68.79721314374448582, -278.7722335525762674, -340.1167290000392427 ) ) ;
#14954=CARTESIAN_POINT ( 'NONE',  ( -41.04906222738272703, -279.8375148345883190, -197.4553193737886261 ) ) ;
#14955=CARTESIAN_POINT ( 'NONE',  ( -35.37162931937074717, -276.0568604820846303, -195.7295285254807311 ) ) ;
#14956=CARTESIAN_POINT ( 'NONE',  ( 26.49290192793644039, -292.9837191468247397, -227.2075566129864228 ) ) ;
#14957=CARTESIAN_POINT ( 'NONE',  ( -79.11532057194287404, -287.6383677775764909, -332.2845840338926564 ) ) ;
#14958=CARTESIAN_POINT ( 'NONE',  ( -90.24533864937700400, -292.9194083385741010, -215.4458629062697241 ) ) ;
#14959=CARTESIAN_POINT ( 'NONE',  ( -72.28397215722968383, -294.4462566618455526, -334.8212685081921336 ) ) ;
#14960=CARTESIAN_POINT ( 'NONE',  ( 35.31681878442596911, -293.1165679105013737, -262.6038851894221011 ) ) ;
#14961=CARTESIAN_POINT ( 'NONE',  ( -110.9394065383886812, -291.9033409344772281, -248.8002710330150364 ) ) ;
#14962=CARTESIAN_POINT ( 'NONE',  ( 35.13272348906826892, -282.0727082826430205, -260.4273368241869093 ) ) ;
#14963=CARTESIAN_POINT ( 'NONE',  ( -114.1064060109667651, -271.6110516640039805, -270.3491600855638239 ) ) ;
#14964=CARTESIAN_POINT ( 'NONE',  ( -20.51062525802773351, -289.4930302992212887, -345.4492248958403025 ) ) ;
#14965=CARTESIAN_POINT ( 'NONE',  ( -24.76237100262590829, -281.0330339411779050, -345.1275879789250212 ) ) ;
#14966=CARTESIAN_POINT ( 'NONE',  ( -26.14344049597411868, -289.2465771672572146, -346.5211027033329287 ) ) ;
#14967=CARTESIAN_POINT ( 'NONE',  ( -7.011593792237876599, -286.7947134366567070, -203.9232042942724945 ) ) ;
#14969=CARTESIAN_POINT ( 'NONE',  ( -32.49014215546316819, -123.7434641620947957, -362.3882418532662086 ) ) ;
#14970=CARTESIAN_POINT ( 'NONE',  ( -88.60724157838485837, -229.4615865740312302, -344.3535732501791813 ) ) ;
#14971=CARTESIAN_POINT ( 'NONE',  ( -93.20689720124428845, -278.4194059840971818, -223.1011745418307726 ) ) ;
#14972=CARTESIAN_POINT ( 'NONE',  ( -6.627414243512323999, -279.3854880942175214, -203.7827179562788160 ) ) ;
#14973=CARTESIAN_POINT ( 'NONE',  ( -21.35503853749595038, -273.9185196053519462, -195.0605805168563904 ) ) ;
#14974=CARTESIAN_POINT ( 'NONE',  ( 86.31154334970720754, 81.21865059938454579, -300.0628701344159026 ) ) ;
#14975=CARTESIAN_POINT ( 'NONE',  ( -98.09673289820428010, -277.7496644967953330, -223.9994142220614890 ) ) ;
#14976=CARTESIAN_POINT ( 'NONE',  ( -77.02237623229856922, -281.6063047001998143, -333.6463898800645325 ) ) ;
#14977=CARTESIAN_POINT ( 'NONE',  ( 21.51614788923746957, -295.9661589534562722, -318.4411793381928533 ) ) ;
#14978=CARTESIAN_POINT ( 'NONE',  ( 2.268601807664912151, -293.0905317938339749, -208.9089070657932155 ) ) ;
#14979=CARTESIAN_POINT ( 'NONE',  ( -68.98538526581214114, -288.1620924613305306, -336.6930158191238434 ) ) ;
#14980=CARTESIAN_POINT ( 'NONE',  ( -0.1020843505969328407, -275.1855965478910093, -203.0666997650090195 ) ) ;
#14981=CARTESIAN_POINT ( 'NONE',  ( -95.60304813716530248, -296.1007189230272729, -314.3659716367945407 ) ) ;
#14985=CARTESIAN_POINT ( 'NONE',  ( -110.6940134173985228, -280.7040620972180136, -252.1764334608224658 ) ) ;
#14986=CARTESIAN_POINT ( 'NONE',  ( -54.57875233172333651, -280.9052261001969555, -199.0548544606908479 ) ) ;
#14987=CARTESIAN_POINT ( 'NONE',  ( 12.31284386041327394, -282.4926524108478247, -212.8424229979267182 ) ) ;
#14988=CARTESIAN_POINT ( 'NONE',  ( 34.16757747435598702, -280.8187364540268049, -286.1671821891202967 ) ) ;
#14989=CARTESIAN_POINT ( 'NONE',  ( -95.14460582801808641, -271.6710503333297311, -224.6497206361564452 ) ) ;
#14992=CARTESIAN_POINT ( 'NONE',  ( 37.78534682813666024, -276.1520850359382848, -254.1717835756720376 ) ) ;
#14994=CARTESIAN_POINT ( 'NONE',  ( 27.38314933737237666, -278.0586348467960534, -308.2516776032041435 ) ) ;
#14995=CARTESIAN_POINT ( 'NONE',  ( -113.4935322293544715, -277.0399404809643897, -277.2596813832041676 ) ) ;
#14998=CARTESIAN_POINT ( 'NONE',  ( -110.1389918356320976, -286.7833694054314151, -250.6978230695078196 ) ) ;
#14999=CARTESIAN_POINT ( 'NONE',  ( -62.84746493801604572, -290.9085685147545064, -201.7895663856133694 ) ) ;
#15000=CARTESIAN_POINT ( 'NONE',  ( 30.04623942745260123, -286.4191271247048576, -233.2076839432773738 ) ) ;
#15002=CARTESIAN_POINT ( 'NONE',  ( -71.90164103808086793, -281.7554848245586641, -335.8102165222308031 ) ) ;
#15003=CARTESIAN_POINT ( 'NONE',  ( -85.25908969992632080, -282.3042897298263938, -326.2118000926590753 ) ) ;
#15004=CARTESIAN_POINT ( 'NONE',  ( 34.78987223875954982, -285.3933027309886938, -251.9152952440694264 ) ) ;
#15005=CARTESIAN_POINT ( 'NONE',  ( 30.70838515815050584, -283.1235094390634686, -297.8623251642928267 ) ) ;
#15006=CARTESIAN_POINT ( 'NONE',  ( 33.84007599325015292, -273.2447717854151392, -246.5719272808927656 ) ) ;
#15007=CARTESIAN_POINT ( 'NONE',  ( -82.78230859198515645, -283.8426834486686516, -209.1267822330590889 ) ) ;
#15008=CARTESIAN_POINT ( 'NONE',  ( -106.5201652567127013, -298.1724354960462051, -299.4667983817611798 ) ) ;
#15009=CARTESIAN_POINT ( 'NONE',  ( -108.5211794547556394, -279.7200118655020447, -253.1306167810067222 ) ) ;
#15010=CARTESIAN_POINT ( 'NONE',  ( -18.66283607850124682, -288.2921875825855409, -197.4984832830887456 ) ) ;
#15013=CARTESIAN_POINT ( 'NONE',  ( 22.81368772070251438, -294.8511037498579412, -224.6162796294288171 ) ) ;
#15014=CARTESIAN_POINT ( 'NONE',  ( -84.27769824464698445, -275.6971742524810338, -328.9259482955554859 ) ) ;
#15015=CARTESIAN_POINT ( 'NONE',  ( -31.84855113190473119, -288.1818026388085627, -347.0554853498662169 ) ) ;
#15016=CARTESIAN_POINT ( 'NONE',  ( 24.01759222698796847, -291.3887566956260002, -229.3552933115682322 ) ) ;
#15017=CARTESIAN_POINT ( 'NONE',  ( -110.8854857240149556, -277.2335365151951123, -270.6232096094690860 ) ) ;
#15018=CARTESIAN_POINT ( 'NONE',  ( -97.08045603927816103, -295.2993886052756238, -226.2698743778591677 ) ) ;
#15019=CARTESIAN_POINT ( 'NONE',  ( -9.556458195699242708, -293.7380232817252477, -202.2685764672799280 ) ) ;
#15020=CARTESIAN_POINT ( 'NONE',  ( 21.27581636871892101, -283.4090924074130839, -223.5744983911110353 ) ) ;
#15021=CARTESIAN_POINT ( 'NONE',  ( 24.31453355230742730, -292.6344332744985195, -315.3410633823395415 ) ) ;
#15022=CARTESIAN_POINT ( 'NONE',  ( 35.92082104460875058, -289.2682972532041958, -279.2517538508241159 ) ) ;
#15023=CARTESIAN_POINT ( 'NONE',  ( -111.5801897380402607, -288.5866415476621683, -286.5666934985757734 ) ) ;
#15025=CARTESIAN_POINT ( 'NONE',  ( -50.84189352776427739, -290.6531517491407044, -342.7535163362921367 ) ) ;
#15027=CARTESIAN_POINT ( 'NONE',  ( -107.1029723889671459, -291.0614100677571514, -292.5732546423507188 ) ) ;
#15029=CARTESIAN_POINT ( 'NONE',  ( -29.00506106599234712, -290.1539274419343428, -346.5623112812566546 ) ) ;
#15030=CARTESIAN_POINT ( 'NONE',  ( -5.613093777918063410, -278.4874904831101503, -202.0112654156020824 ) ) ;
#15032=CARTESIAN_POINT ( 'NONE',  ( 32.00426472833874669, -280.7886414897344025, -236.8186949681834506 ) ) ;
#15033=CARTESIAN_POINT ( 'NONE',  ( 25.21597841165944232, -284.9922498285788492, -228.8963127811026652 ) ) ;
#15034=CARTESIAN_POINT ( 'NONE',  ( 36.36325840924525465, -279.8120422741844777, -279.6356725192413251 ) ) ;
#15035=CARTESIAN_POINT ( 'NONE',  ( -68.92674225723072823, -283.6367567202963187, -202.3222366353230655 ) ) ;
#15036=CARTESIAN_POINT ( 'NONE',  ( 139.3042674286450051, 178.0593505315339655, -238.4361928449195602 ) ) ;
#15037=CARTESIAN_POINT ( 'NONE',  ( -110.7785769561892408, -276.7698706796314809, -291.0911173873932398 ) ) ;
#15038=CARTESIAN_POINT ( 'NONE',  ( -101.1695466135648189, -282.9095998109747825, -312.9711149987672343 ) ) ;
#15039=CARTESIAN_POINT ( 'NONE',  ( 94.93239848020441229, -300.6892790076082065, -197.1041445370088354 ) ) ;
#15040=CARTESIAN_POINT ( 'NONE',  ( -33.48680555501966438, -293.7015803428286631, -196.6492336337761913 ) ) ;
#15041=CARTESIAN_POINT ( 'NONE',  ( -55.21354456981067926, -275.2518910279451347, -196.0697761752051633 ) ) ;
#15042=CARTESIAN_POINT ( 'NONE',  ( 5.405729127621107466, -276.1225488142885069, -329.6244407452855967 ) ) ;
#15043=CARTESIAN_POINT ( 'NONE',  ( -23.11516070898414199, -296.8704908374231195, -344.0524863797014063 ) ) ;
#15044=CARTESIAN_POINT ( 'NONE',  ( -6.917972340403921727, -288.8304841365395532, -341.1100513044441982 ) ) ;
#15045=CARTESIAN_POINT ( 'NONE',  ( 30.73491404735966981, -279.2020239408659563, -237.4551676188944782 ) ) ;
#15046=CARTESIAN_POINT ( 'NONE',  ( -25.01934905682688637, -292.0384784206648874, -194.3534889670114012 ) ) ;
#15047=CARTESIAN_POINT ( 'NONE',  ( -81.86261354133968382, -290.4875955915459826, -212.1480359353932670 ) ) ;
#15048=CARTESIAN_POINT ( 'NONE',  ( -64.89313275815500504, -293.4118216278505429, -340.1311137358343331 ) ) ;
#15051=CARTESIAN_POINT ( 'NONE',  ( -101.1743930792914057, -290.5466534028199135, -234.7132238697029152 ) ) ;
#15053=CARTESIAN_POINT ( 'NONE',  ( -46.48938434906518324, -286.8799970140468076, -194.1434029421205878 ) ) ;
#15054=CARTESIAN_POINT ( 'NONE',  ( -109.1418805571601069, -293.0519495502701943, -270.3937649182068412 ) ) ;
#15055=CARTESIAN_POINT ( 'NONE',  ( 21.18047541082637508, -293.2826326623358568, -320.0398376101054509 ) ) ;
#15056=CARTESIAN_POINT ( 'NONE',  ( 35.14725911861896179, -283.1793510136896543, -294.9931703800187961 ) ) ;
#15057=CARTESIAN_POINT ( 'NONE',  ( -110.3904368893083188, -284.3782675227793106, -270.9071810373341691 ) ) ;
#15058=CARTESIAN_POINT ( 'NONE',  ( 31.73096269163791661, -277.2013220914643057, -295.6130954307375873 ) ) ;
#15059=CARTESIAN_POINT ( 'NONE',  ( -8.620803034927837061, -292.6945637510834217, -339.2731911420747792 ) ) ;
#15060=CARTESIAN_POINT ( 'NONE',  ( 25.70887004303792267, -274.8608684744641550, -307.9344609968768509 ) ) ;
#15063=CARTESIAN_POINT ( 'NONE',  ( -44.79780244011147516, -294.8106668546647597, -347.0314196467380725 ) ) ;
#15064=CARTESIAN_POINT ( 'NONE',  ( 34.41089179808677301, -289.2154550940693412, -250.5399234762938363 ) ) ;
#15065=CARTESIAN_POINT ( 'NONE',  ( -79.29632203766676923, -296.6839561113782224, -334.5584871624771495 ) ) ;
#15066=CARTESIAN_POINT ( 'NONE',  ( -42.68985327603825652, -286.6343449060184412, -197.4424398264602303 ) ) ;
#15067=CARTESIAN_POINT ( 'NONE',  ( -70.21118042624624422, -276.5334392491919857, -339.7471019975104127 ) ) ;
#15068=CARTESIAN_POINT ( 'NONE',  ( 8.851551046606893181, -295.0884493974060661, -331.8387263630948496 ) ) ;
#15069=CARTESIAN_POINT ( 'NONE',  ( -68.86533399736563865, -287.6017585140245387, -339.2706389777469553 ) ) ;
#15071=CARTESIAN_POINT ( 'NONE',  ( -112.5807388420076194, -297.0897328479682074, -254.0259377198101447 ) ) ;
#15072=CARTESIAN_POINT ( 'NONE',  ( -34.86081443189331708, -292.4174554811343683, -197.3821299585684699 ) ) ;
#15073=DIRECTION ( 'NONE',  ( 0.000000000000000000, 0.000000000000000000, -1.000000000000000000 ) ) ;
#15075=CARTESIAN_POINT ( 'NONE',  ( 122.1069166414435188, 147.2784711290201471, -260.4370888796501049 ) ) ;
#15077=CARTESIAN_POINT ( 'NONE',  ( 32.07319419917863712, -288.6620186997694191, -238.5436092288638008 ) ) ;
#15078=CARTESIAN_POINT ( 'NONE',  ( -19.05039376806006857, -289.7666405000204009, -190.3683826091709363 ) ) ;
#15080=CARTESIAN_POINT ( 'NONE',  ( -11.53573798968777808, -279.7280760774544319, -197.8665084577066864 ) ) ;
#15081=CARTESIAN_POINT ( 'NONE',  ( -10.28983966323379207, -284.6985922698972900, -340.1887215999643104 ) ) ;
#15082=CARTESIAN_POINT ( 'NONE',  ( -78.19201225635383423, -284.0889241552297904, -205.7866780614738786 ) ) ;
#15083=CARTESIAN_POINT ( 'NONE',  ( 8.854837899617368890, -286.4927039141430782, -328.7322929675459591 ) ) ;
#15084=CARTESIAN_POINT ( 'NONE',  ( 0.5567041505140671864, -276.4120096259011916, -204.7410773755840410 ) ) ;
#15085=CARTESIAN_POINT ( 'NONE',  ( -39.17615333602782357, -298.5208969413874911, -197.3101936461422099 ) ) ;
#15086=CARTESIAN_POINT ( 'NONE',  ( 12.67833886840204194, -293.0221489522724596, -324.2754369872645839 ) ) ;
#15087=CARTESIAN_POINT ( 'NONE',  ( -35.34699757052139546, -280.7279509746610415, -193.4758061816777115 ) ) ;
#15088=CARTESIAN_POINT ( 'NONE',  ( 26.76675462052174836, -276.0300280861304714, -305.3824898953262732 ) ) ;
#15089=CARTESIAN_POINT ( 'NONE',  ( -67.34054376307322798, -278.9966276392759141, -203.6844449848367162 ) ) ;
#15090=CARTESIAN_POINT ( 'NONE',  ( 33.42299129710904992, -276.2528072928744791, -240.6630493985697115 ) ) ;
#15091=CARTESIAN_POINT ( 'NONE',  ( -107.2997974446115279, -277.0681046019389555, -301.9126302051150788 ) ) ;
#15092=CARTESIAN_POINT ( 'NONE',  ( -114.1313154040836650, -273.2851564102892326, -284.1365878591568617 ) ) ;
#15093=CARTESIAN_POINT ( 'NONE',  ( 8.501874767114017573, -274.4246346221747217, -329.7838799706123041 ) ) ;
#15095=CARTESIAN_POINT ( 'NONE',  ( -108.3478281756182611, -298.3398420032713148, -241.9923298175449986 ) ) ;
#15097=CARTESIAN_POINT ( 'NONE',  ( 181.0595704366054690, 252.2700355933461651, -164.3583243123303532 ) ) ;
#15098=CARTESIAN_POINT ( 'NONE',  ( 11.32905525087031329, -287.8249880494316244, -215.4715456183801336 ) ) ;
#15099=CARTESIAN_POINT ( 'NONE',  ( -70.64263240357119855, -287.3791606541255987, -202.0601521967194287 ) ) ;
#15100=CARTESIAN_POINT ( 'NONE',  ( -5.747091079040602679, -285.8274415608531740, -204.4255927919825240 ) ) ;
#15101=CARTESIAN_POINT ( 'NONE',  ( -91.87437193537228097, -277.6573801885731427, -220.6355901185366122 ) ) ;
#15102=CARTESIAN_POINT ( 'NONE',  ( -109.2306541176174051, -286.6529267508993257, -251.8450769067680994 ) ) ;
#15103=CARTESIAN_POINT ( 'NONE',  ( -109.8104306148581912, -277.2068540914880259, -256.9823715791741847 ) ) ;
#15104=CARTESIAN_POINT ( 'NONE',  ( -70.66151415100436850, -278.8163666521174378, -335.8670984182563188 ) ) ;
#15105=CARTESIAN_POINT ( 'NONE',  ( 32.91746112377272482, -275.7775925708898512, -250.1394727498181680 ) ) ;
#15106=CARTESIAN_POINT ( 'NONE',  ( 38.28046640983761506, -286.5047333481776377, -282.9019149496307364 ) ) ;
#15107=CARTESIAN_POINT ( 'NONE',  ( 15.04375573756397344, -281.5713180107804874, -214.0752013055139287 ) ) ;
#15108=CARTESIAN_POINT ( 'NONE',  ( 34.53225460434799743, -282.3923296939545935, -297.8140146280107388 ) ) ;
#15112=FACE_OUTER_BOUND ( 'NONE', #7241, .T. ) ;
#15113=CARTESIAN_POINT ( 'NONE',  ( -92.67423654594335858, -291.6945329200743799, -322.1920477383625894 ) ) ;
#15114=CARTESIAN_POINT ( 'NONE',  ( -75.43277900722347340, -288.2339815521284550, -336.7114607301139699 ) ) ;
#15115=CARTESIAN_POINT ( 'NONE',  ( -67.88659909682871785, -297.0465831497848512, -340.1712144159924378 ) ) ;
#15116=CARTESIAN_POINT ( 'NONE',  ( -37.81332025501148308, -297.2432611803557165, -197.2011610251920501 ) ) ;
#15117=CARTESIAN_POINT ( 'NONE',  ( -61.64848547805958390, -291.0931490998294180, -197.3496199144815364 ) ) ;
#15118=CARTESIAN_POINT ( 'NONE',  ( 25.55243892172937592, -285.5078758314507468, -231.9549332623005000 ) ) ;
#15119=CARTESIAN_POINT ( 'NONE',  ( -18.35607478536340409, -290.0072445144078301, -341.3130515415115269 ) ) ;
#15120=CARTESIAN_POINT ( 'NONE',  ( -110.4683760289727132, -293.2662352645559167, -253.7030783399848985 ) ) ;
#15121=CARTESIAN_POINT ( 'NONE',  ( -45.77491134458503552, -291.1590929135921328, -344.9372332756022956 ) ) ;
#15122=CARTESIAN_POINT ( 'NONE',  ( -38.90812818273636253, -287.0716063446362227, -345.5114655092765474 ) ) ;
#15123=CARTESIAN_POINT ( 'NONE',  ( -38.03165292124556629, -291.0609193960547714, -345.3705491469568756 ) ) ;
#15124=CARTESIAN_POINT ( 'NONE',  ( -106.3915783605032601, -285.1678883361105932, -294.9153939111548084 ) ) ;
#15125=CARTESIAN_POINT ( 'NONE',  ( -58.44887042212440065, -293.7800610208776106, -198.2187879246360751 ) ) ;
#15127=CARTESIAN_POINT ( 'NONE',  ( 133.0872704186301405, -299.5541904835127980, -188.7068768330456123 ) ) ;
#15128=CARTESIAN_POINT ( 'NONE',  ( -95.67911939684735501, -275.1865666471322811, -222.6424180280208702 ) ) ;
#15129=CARTESIAN_POINT ( 'NONE',  ( 35.68165889153419101, -280.6901700420580141, -265.8677045765517732 ) ) ;
#15130=CARTESIAN_POINT ( 'NONE',  ( -77.21131527937788519, -281.5860396752066208, -333.9474617813671102 ) ) ;
#15131=CARTESIAN_POINT ( 'NONE',  ( -65.55374574031428381, -294.6089562854335782, -341.8472586566103928 ) ) ;
#15132=CARTESIAN_POINT ( 'NONE',  ( -38.07015221690794249, -272.2827592662044935, -196.3513660982877980 ) ) ;
#15133=CARTESIAN_POINT ( 'NONE',  ( -5.686042623816032204, -274.7124529648054363, -337.7489897319943566 ) ) ;
#15134=CARTESIAN_POINT ( 'NONE',  ( -97.29466702524970856, -298.4568777370442376, -227.8536452406141848 ) ) ;
#15136=CARTESIAN_POINT ( 'NONE',  ( -55.17833286309119956, -272.4018052091549862, -196.0613143222341250 ) ) ;
#15137=CARTESIAN_POINT ( 'NONE',  ( -103.7286542139609651, -294.3051287464018628, -307.4382704674184197 ) ) ;
#15138=CARTESIAN_POINT ( 'NONE',  ( 24.93551944878662496, -295.5157472086812618, -309.6604822016483354 ) ) ;
#15140=CARTESIAN_POINT ( 'NONE',  ( -6.687959855693156541, -295.4419057846418468, -336.7911558780933206 ) ) ;
#15143=CARTESIAN_POINT ( 'NONE',  ( -108.6759548807474545, -282.2595898787317310, -294.6475524849048497 ) ) ;
#15144=CARTESIAN_POINT ( 'NONE',  ( -109.1421302913753664, -296.3773796871216746, -283.6098271359936689 ) ) ;
#15145=CARTESIAN_POINT ( 'NONE',  ( -114.1518519013656885, -284.6286021544469804, -264.2482390723681647 ) ) ;
#15146=CARTESIAN_POINT ( 'NONE',  ( -30.32383195700539247, -284.8841808350481983, -345.5945129873040855 ) ) ;
#15147=AXIS2_PLACEMENT_3D ( 'NONE', #19397, #89947, #33596 ) ;
#15148=CARTESIAN_POINT ( 'NONE',  ( 22.97796748170735626, -286.5784999961942958, -222.5145695767751590 ) ) ;
#15149=CARTESIAN_POINT ( 'NONE',  ( -38.91111842682269639, -290.0322565442247083, -195.5442391632657007 ) ) ;
#15150=CARTESIAN_POINT ( 'NONE',  ( -11.55389753143429843, -279.5766811162470162, -197.9232906108013026 ) ) ;
#15151=CARTESIAN_POINT ( 'NONE',  ( 21.31550574532286291, -278.4094976428775681, -223.6242672951989618 ) ) ;
#15153=CARTESIAN_POINT ( 'NONE',  ( 23.87367499471782750, -285.7872063392975406, -229.7745261804603558 ) ) ;
#15155=CARTESIAN_POINT ( 'NONE',  ( -113.6976929224262136, -289.5692559804612074, -262.6542961799540308 ) ) ;
#15158=CARTESIAN_POINT ( 'NONE',  ( -111.1664840662578797, -280.2266880505036397, -250.5999620905804477 ) ) ;
#15159=CARTESIAN_POINT ( 'NONE',  ( -55.69461930861432108, -293.3073680560329990, -343.4472121274324081 ) ) ;
#15160=CARTESIAN_POINT ( 'NONE',  ( -4.334214791337673844, -280.1663689781372568, -205.2120293380274347 ) ) ;
#15161=CARTESIAN_POINT ( 'NONE',  ( -69.52598625362830376, -295.6308246069863799, -340.3267605181873705 ) ) ;
#15162=CARTESIAN_POINT ( 'NONE',  ( 33.51256270610736010, -285.2938291448624000, -244.1125440293015458 ) ) ;
#15164=CARTESIAN_POINT ( 'NONE',  ( -85.53946260179677097, -281.3861835382718368, -212.8305810109754361 ) ) ;
#15165=CARTESIAN_POINT ( 'NONE',  ( -108.7036198770296238, -295.8273178367575156, -253.9025378886643409 ) ) ;
#15168=CARTESIAN_POINT ( 'NONE',  ( -79.28039158902841166, -285.6012269008483599, -332.1105548955749782 ) ) ;
#15170=CARTESIAN_POINT ( 'NONE',  ( 35.78497577281001440, -290.8380690714490129, -253.7030783399848985 ) ) ;
#15171=CARTESIAN_POINT ( 'NONE',  ( -27.00809219693016772, -273.3773799382550465, -194.1673019692075286 ) ) ;
#15172=CARTESIAN_POINT ( 'NONE',  ( -83.82740409146008176, -291.2261186226832592, -214.0754241384555883 ) ) ;
#15173=CARTESIAN_POINT ( 'NONE',  ( 36.38051391880737384, -283.0485808111613437, -268.5473783609551219 ) ) ;
#15174=CARTESIAN_POINT ( 'NONE',  ( -32.66042078798253812, -275.7122325980164419, -196.6970725281209127 ) ) ;
#15175=CARTESIAN_POINT ( 'NONE',  ( -60.96410810636794508, -284.9537285270282041, -342.8622135639787984 ) ) ;
#15176=CARTESIAN_POINT ( 'NONE',  ( 17.89361162317399945, -281.0330107919604075, -318.6952761040914766 ) ) ;
#15177=CARTESIAN_POINT ( 'NONE',  ( -110.8524918838389226, -280.7440893845216010, -255.4249316866856248 ) ) ;
#15178=CARTESIAN_POINT ( 'NONE',  ( -114.3417789856397206, -272.7546669925150127, -267.4957702519898248 ) ) ;
#15180=CARTESIAN_POINT ( 'NONE',  ( -52.54354444183928052, -273.6960529915692177, -194.8222157423174963 ) ) ;
#15181=CARTESIAN_POINT ( 'NONE',  ( 36.72557489202645797, -295.3696400451231625, -262.4245545433521443 ) ) ;
#15184=CARTESIAN_POINT ( 'NONE',  ( 35.18033417861960999, -291.9735157018828886, -292.4671728409064144 ) ) ;
#15185=CARTESIAN_POINT ( 'NONE',  ( 19.05034733944065906, -274.4020271799920465, -223.9076420708660464 ) ) ;
#15186=CARTESIAN_POINT ( 'NONE',  ( -1.149923282487198328, -294.0436351797982297, -203.1832716152183309 ) ) ;
#15187=CARTESIAN_POINT ( 'NONE',  ( 10.64812456238590066, -284.9090924074130271, -330.4860931364851808 ) ) ;
#15188=CARTESIAN_POINT ( 'NONE',  ( -69.47069151011361043, -292.8437452892238753, -200.8073884647353680 ) ) ;
#15189=CARTESIAN_POINT ( 'NONE',  ( 9.138077453083853996, -290.4123875631011060, -329.0097215410813192 ) ) ;
#15190=CARTESIAN_POINT ( 'NONE',  ( 30.81377120221815247, -273.9582843033544464, -301.2619294799239356 ) ) ;
#15191=CARTESIAN_POINT ( 'NONE',  ( -83.88849966740357900, -279.6168580128189092, -328.5196936287024982 ) ) ;
#15192=CARTESIAN_POINT ( 'NONE',  ( 24.10814507329684275, -292.2063990126723638, -312.4658663561411345 ) ) ;
#15193=CARTESIAN_POINT ( 'NONE',  ( 37.56973689817415618, -283.2641227162248470, -258.6821395268172523 ) ) ;
#15195=CARTESIAN_POINT ( 'NONE',  ( -42.93877096930648207, -282.7913153760666205, -343.2175393619461374 ) ) ;
#15196=CARTESIAN_POINT ( 'NONE',  ( -36.76872702404064341, -281.1388620501670061, -193.6593761586896676 ) ) ;
#15197=CARTESIAN_POINT ( 'NONE',  ( -44.39800356312578344, -281.9343242565125252, -346.6914404667514873 ) ) ;
#15198=CARTESIAN_POINT ( 'NONE',  ( -67.60478041881619049, -278.3808782455269011, -340.9087344180882724 ) ) ;
#15200=CARTESIAN_POINT ( 'NONE',  ( 10.11018211553916935, -277.9319559669725663, -330.1866714896522694 ) ) ;
#15202=CARTESIAN_POINT ( 'NONE',  ( -105.5937364680635966, -293.2662352645559167, -254.8156830097664738 ) ) ;
#15205=CARTESIAN_POINT ( 'NONE',  ( -111.4008184333346065, -274.6950462627561365, -259.2695261873302002 ) ) ;
#15207=CARTESIAN_POINT ( 'NONE',  ( -77.25617295882872781, -275.6098506058735893, -333.4987112014621857 ) ) ;
#15208=CARTESIAN_POINT ( 'NONE',  ( -112.8044270791010604, -292.1939099488014335, -279.7022446076493907 ) ) ;
#15209=CARTESIAN_POINT ( 'NONE',  ( 28.48273147314468190, -293.3318477017017472, -302.2746340421704758 ) ) ;
#15210=CARTESIAN_POINT ( 'NONE',  ( -12.24972785872560621, -288.2420591111903150, -343.1487780468973483 ) ) ;
#15211=CARTESIAN_POINT ( 'NONE',  ( 129.4467878515196162, -299.5541904835127980, -192.3225193827704516 ) ) ;
#15212=CARTESIAN_POINT ( 'NONE',  ( 25.22169536677001034, -292.7117216417075838, -314.2522465222793357 ) ) ;
#15213=CARTESIAN_POINT ( 'NONE',  ( -56.54650048823933162, -281.7037129241570597, -341.6185109766022947 ) ) ;
#15214=CARTESIAN_POINT ( 'NONE',  ( -39.97847150189620180, -290.9459225210188720, -344.5998935871107847 ) ) ;
#15215=CARTESIAN_POINT ( 'NONE',  ( -107.1832547316018918, -283.3433181230396940, -246.6883776761474394 ) ) ;
#15216=CARTESIAN_POINT ( 'NONE',  ( -26.65462342375412064, -284.2286824502753575, -343.1247307671146132 ) ) ;
#15217=CARTESIAN_POINT ( 'NONE',  ( -109.6398879997262270, -291.1649302301790385, -296.3215886702050170 ) ) ;
#15218=CARTESIAN_POINT ( 'NONE',  ( 35.58089727719877260, -281.9851412922354257, -265.8574273658376796 ) ) ;
#15219=CARTESIAN_POINT ( 'NONE',  ( -30.64104909141789079, -293.7641350407864707, -346.6704227500508750 ) ) ;
#15220=CARTESIAN_POINT ( 'NONE',  ( 16.17937307715149942, -287.5914534149048336, -215.2280648914523624 ) ) ;
#15221=CARTESIAN_POINT ( 'NONE',  ( 38.22855990177499308, -287.8636958294777060, -255.9159560789599368 ) ) ;
#15222=CARTESIAN_POINT ( 'NONE',  ( -93.25646967994852332, -285.3852928549603689, -223.4299071470096294 ) ) ;
#15225=CARTESIAN_POINT ( 'NONE',  ( -39.05576025648635863, -296.9338577699517714, -346.1065302623649131 ) ) ;
#15226=CARTESIAN_POINT ( 'NONE',  ( -92.35411657558167065, -294.5039483130847771, -323.5300215732144125 ) ) ;
#15227=CARTESIAN_POINT ( 'NONE',  ( -100.7926649505992032, -277.1098693812487568, -307.0332514468245222 ) ) ;
#15228=CARTESIAN_POINT ( 'NONE',  ( -36.53361470600247429, -297.4106111465627009, -193.4631366652685358 ) ) ;
#15229=CARTESIAN_POINT ( 'NONE',  ( 27.76159930737323123, -292.4992830571406444, -304.9993451199967467 ) ) ;
#15230=CARTESIAN_POINT ( 'NONE',  ( -16.37477079689389825, -276.0868861471752780, -199.3262642550542125 ) ) ;
#15231=CARTESIAN_POINT ( 'NONE',  ( -90.76194001227179342, -295.5218988998871623, -219.0603444925297083 ) ) ;
#15232=CARTESIAN_POINT ( 'NONE',  ( 21.65473534918080034, -295.3661067126975013, -314.0251891018666583 ) ) ;
#15233=CARTESIAN_POINT ( 'NONE',  ( 24.69614967220579516, -295.1702020146665859, -309.5145514576460073 ) ) ;
#15235=CARTESIAN_POINT ( 'NONE',  ( -111.0849887327953667, -294.7393583508400638, -255.7363352942988968 ) ) ;
#15236=CARTESIAN_POINT ( 'NONE',  ( -112.3426482175930232, -274.5879229896262359, -267.5880413896982759 ) ) ;
#15237=CARTESIAN_POINT ( 'NONE',  ( -70.06685188145638676, -290.4354718463557674, -335.8919867721832588 ) ) ;
#15238=CARTESIAN_POINT ( 'NONE',  ( -93.09579115647140668, -296.2152653224621872, -317.5352197962346850 ) ) ;
#15239=CARTESIAN_POINT ( 'NONE',  ( -110.2299268573743234, -280.2868485705914168, -289.5353831041932722 ) ) ;
#15240=CARTESIAN_POINT ( 'NONE',  ( -36.73950691828656545, -278.7444045972972617, -193.8436745294311550 ) ) ;
#15241=CARTESIAN_POINT ( 'NONE',  ( 35.96295379401282588, -275.1931366905004666, -293.5934338363402389 ) ) ;
#15242=CARTESIAN_POINT ( 'NONE',  ( -33.44482177080126206, -281.0825913060816106, -344.7118733701401538 ) ) ;
#15243=CARTESIAN_POINT ( 'NONE',  ( -111.3044303039521026, -277.1843491475054293, -251.9785694830478633 ) ) ;
#15244=CARTESIAN_POINT ( 'NONE',  ( -50.59085277116972179, -277.8831487169188108, -196.3713323494931444 ) ) ;
#15245=CARTESIAN_POINT ( 'NONE',  ( -98.85119200914509463, -295.7917788416601752, -230.0468487854578541 ) ) ;
#15246=CARTESIAN_POINT ( 'NONE',  ( -0.6409153747703357773, -276.5398619184994118, -204.9397115528984727 ) ) ;
#15248=CARTESIAN_POINT ( 'NONE',  ( -104.5259899121446239, -289.0225677856435595, -236.1187607721205097 ) ) ;
#15249=CARTESIAN_POINT ( 'NONE',  ( -37.50159019729269971, -289.0540657626553980, -347.3740238018522177 ) ) ;
#15250=CARTESIAN_POINT ( 'NONE',  ( 26.92160825705013494, -277.0297592119269439, -231.2712117033388495 ) ) ;
#15251=CARTESIAN_POINT ( 'NONE',  ( -96.16592741527880150, -271.1910895173010658, -223.8346638131558564 ) ) ;
#15252=CARTESIAN_POINT ( 'NONE',  ( -112.9798667870211659, -283.5761080244857908, -284.1822007142310440 ) ) ;
#15253=CARTESIAN_POINT ( 'NONE',  ( 129.9467878515196162, -299.5541904835127980, -190.0176033293537898 ) ) ;
#15254=CARTESIAN_POINT ( 'NONE',  ( -108.4072419239234364, -282.2401706353770692, -294.4920533174262118 ) ) ;
#15256=CARTESIAN_POINT ( 'NONE',  ( 35.10835770291462410, -292.1918442871239563, -258.5299957570583160 ) ) ;
#15257=CARTESIAN_POINT ( 'NONE',  ( -111.6266230412442440, -282.6848041490763421, -270.8949300268375850 ) ) ;
#15260=CARTESIAN_POINT ( 'NONE',  ( 23.44011677327116416, -290.9534921397819289, -226.4010016420293141 ) ) ;
#15261=CARTESIAN_POINT ( 'NONE',  ( 38.72214182766492030, -279.9552676791909107, -264.2783802516528908 ) ) ;
#15262=CARTESIAN_POINT ( 'NONE',  ( -109.2613332816082590, -279.9355551561741891, -286.9702070352231544 ) ) ;
#15263=CARTESIAN_POINT ( 'NONE',  ( -110.7231671646470659, -285.4794281973779562, -292.3877419741945118 ) ) ;
#15264=CARTESIAN_POINT ( 'NONE',  ( -59.97862926585872856, -285.7504573797669991, -200.9596090709286784 ) ) ;
#15265=CARTESIAN_POINT ( 'NONE',  ( -61.97006126762443046, -278.8038369874677755, -339.7609340238977325 ) ) ;
#15266=CARTESIAN_POINT ( 'NONE',  ( -96.21687980577205224, -278.7473453197708295, -313.8138406829186806 ) ) ;
#15268=CARTESIAN_POINT ( 'NONE',  ( -82.10319740870546923, -287.4423929183736846, -210.1181951469412468 ) ) ;
#15271=CARTESIAN_POINT ( 'NONE',  ( -108.3758626312435354, -296.0059437428294586, -300.2169273489993770 ) ) ;
#15273=CARTESIAN_POINT ( 'NONE',  ( -59.14603817337341951, -291.3154852591933945, -341.8043035169222890 ) ) ;
#15275=CARTESIAN_POINT ( 'NONE',  ( -2.602324593224680793, -279.1233781216987495, -342.4248175857292154 ) ) ;
#15276=CARTESIAN_POINT ( 'NONE',  ( -73.60728612800370740, -278.5027566370227987, -202.7718266797550086 ) ) ;
#15277=CARTESIAN_POINT ( 'NONE',  ( 38.70227000252714333, -292.0232930154083419, -276.0004507890507170 ) ) ;
#15279=CARTESIAN_POINT ( 'NONE',  ( 33.69247261578643560, -288.8154876329008403, -250.7434204568437224 ) ) ;
#15280=CARTESIAN_POINT ( 'NONE',  ( -39.75644186291612669, -281.7815878370878977, -196.3744897734738117 ) ) ;
#15281=CARTESIAN_POINT ( 'NONE',  ( 0.4438376529203304499, -289.9845874673037542, -336.8352177782438162 ) ) ;
#15282=CARTESIAN_POINT ( 'NONE',  ( -74.77346948222938749, -285.5501706056037392, -335.4115457415587116 ) ) ;
#15283=CARTESIAN_POINT ( 'NONE',  ( -72.83879534774986553, -277.6758520821545062, -338.7055825328710057 ) ) ;
#15285=CARTESIAN_POINT ( 'NONE',  ( -71.19139132135998693, -295.6232275710356134, -203.8183655436061201 ) ) ;
#15286=CARTESIAN_POINT ( 'NONE',  ( 38.00696136140724235, -291.5600222558498444, -264.7136931131582287 ) ) ;
#15287=CARTESIAN_POINT ( 'NONE',  ( -95.90442668975327933, -279.0599880909725243, -220.3467968669700383 ) ) ;
#15288=CARTESIAN_POINT ( 'NONE',  ( -27.14354467667562432, -276.0434319117055111, -196.7779845342168699 ) ) ;
#15290=CARTESIAN_POINT ( 'NONE',  ( -95.95921662488163406, -292.4090924074130839, -317.1477375740089997 ) ) ;
#15291=CARTESIAN_POINT ( 'NONE',  ( -13.36076094935486402, -272.5992579032717913, -198.2577992766572947 ) ) ;
#15293=CARTESIAN_POINT ( 'NONE',  ( -34.30449879329485441, -279.5989798356156939, -197.3501814333233710 ) ) ;
#15294=CARTESIAN_POINT ( 'NONE',  ( 38.34587447068880550, -276.9098398718295471, -282.5012231946375323 ) ) ;
#15295=CARTESIAN_POINT ( 'NONE',  ( -39.20126651060222400, -299.4536711487753564, -196.7828771459608106 ) ) ;
#15296=CARTESIAN_POINT ( 'NONE',  ( -110.8860107189336759, -283.3334469468297812, -292.4080287477763704 ) ) ;
#15297=CARTESIAN_POINT ( 'NONE',  ( 32.36115072820064142, -289.6391468290395323, -295.2506056222009647 ) ) ;
#15298=CARTESIAN_POINT ( 'NONE',  ( -109.2044732964808134, -298.3991135533725014, -244.7008454915571463 ) ) ;
#15299=CARTESIAN_POINT ( 'NONE',  ( -37.62169158028348903, -299.2537886864762413, -193.7587007532200971 ) ) ;
#15300=CARTESIAN_POINT ( 'NONE',  ( 2.568612614507656655, -296.5163127457378209, -333.7249134376760935 ) ) ;
#15301=CARTESIAN_POINT ( 'NONE',  ( -6.521108790400147015, -280.6463450114713964, -338.5669586333523853 ) ) ;
#15302=CARTESIAN_POINT ( 'NONE',  ( -32.56106000304422565, -272.1327900334985088, -195.8567510946501784 ) ) ;
#15303=CARTESIAN_POINT ( 'NONE',  ( -78.11181243102357996, -287.1138372120078657, -205.9853589015050375 ) ) ;
#15304=CARTESIAN_POINT ( 'NONE',  ( -61.36924932555739076, -288.2920254633450554, -339.6207956664441667 ) ) ;
#15305=CARTESIAN_POINT ( 'NONE',  ( -108.6012104099982309, -267.5897348884550979, -306.9379130596528285 ) ) ;
#15307=CARTESIAN_POINT ( 'NONE',  ( 35.38135276139608720, -286.4240771481159982, -293.8124264979344389 ) ) ;
#15308=CARTESIAN_POINT ( 'NONE',  ( 28.24489232128960481, -287.6535754220393528, -302.4623076420973575 ) ) ;
#15310=CARTESIAN_POINT ( 'NONE',  ( -111.4262223471554734, -285.8832941003722681, -250.3377617016133172 ) ) ;
#15311=CARTESIAN_POINT ( 'NONE',  ( -11.24252134828827820, -277.0357179091452053, -338.5587744950851743 ) ) ;
#15312=CARTESIAN_POINT ( 'NONE',  ( 20.15609093970152443, -291.7823411424012079, -219.5919233574116163 ) ) ;
#15313=CARTESIAN_POINT ( 'NONE',  ( 35.22872891725126010, -281.8805532111661023, -244.7689692592749964 ) ) ;
#15314=CARTESIAN_POINT ( 'NONE',  ( -1.478564221311180482, -282.0390073533935720, -203.0072521920707231 ) ) ;
#15315=CARTESIAN_POINT ( 'NONE',  ( -98.02513364858326383, -284.2524103414684191, -317.7242385281491579 ) ) ;
#15316=CARTESIAN_POINT ( 'NONE',  ( -11.73971030273082228, -280.7280505131478208, -201.9217884051330145 ) ) ;
#15317=CARTESIAN_POINT ( 'NONE',  ( -89.88738572736605192, -230.7286653867029713, -347.9689446550020193 ) ) ;
#15318=CARTESIAN_POINT ( 'NONE',  ( -81.89087134799066803, -279.6609526076622387, -330.4893124272986142 ) ) ;
#15319=CARTESIAN_POINT ( 'NONE',  ( -49.19496325650769109, -154.3339921397289913, -364.3446390947307805 ) ) ;
#15320=CARTESIAN_POINT ( 'NONE',  ( -106.7427607202974542, -259.6958249236880647, -315.6408438834064327 ) ) ;
#15321=CARTESIAN_POINT ( 'NONE',  ( -85.40857260003362228, -272.5650094348158063, -215.1376661235696588 ) ) ;
#15322=CARTESIAN_POINT ( 'NONE',  ( 15.43191736720857499, -293.8374305555566934, -326.3474752454189343 ) ) ;
#15323=CARTESIAN_POINT ( 'NONE',  ( 85.24291059917956659, 81.26895831550152138, -298.9807373495123102 ) ) ;
#15325=CARTESIAN_POINT ( 'NONE',  ( -52.43185771060288403, -272.5477438386967606, -195.3031254171106923 ) ) ;
#15326=CARTESIAN_POINT ( 'NONE',  ( -95.59447479657197277, -288.3203665069697195, -315.6921891144242522 ) ) ;
#15327=CARTESIAN_POINT ( 'NONE',  ( -98.18235092230905536, -297.8293001002335814, -312.8967582406389170 ) ) ;
#15329=CARTESIAN_POINT ( 'NONE',  ( 20.75756271806354292, -289.4971424093940300, -315.3894901371530750 ) ) ;
#15330=ORIENTED_EDGE ( 'NONE', *, *, #72825, .T. ) ;
#15331=CARTESIAN_POINT ( 'NONE',  ( -5.883131775773463801, -295.5898353717196301, -340.3838192367417719 ) ) ;
#15332=CARTESIAN_POINT ( 'NONE',  ( 6.959264756027824461, -287.1659062529643620, -212.1988963803346167 ) ) ;
#15333=CARTESIAN_POINT ( 'NONE',  ( -29.85532486723949219, -273.0651550450975265, -194.0365040302886257 ) ) ;
#15334=CARTESIAN_POINT ( 'NONE',  ( 33.17215089936051697, -293.9651387880358584, -239.8331695859829722 ) ) ;
#15335=CARTESIAN_POINT ( 'NONE',  ( 37.36068917164182324, -293.8139545025637744, -251.9469946960184927 ) ) ;
#15336=CARTESIAN_POINT ( 'NONE',  ( -55.01440978826175865, -291.9851717417379859, -199.5326255677821905 ) ) ;
#15338=CARTESIAN_POINT ( 'NONE',  ( -52.28521652858497504, -275.7825512789535765, -196.2401175497192582 ) ) ;
#15339=CARTESIAN_POINT ( 'NONE',  ( 39.22579307701682438, -274.3933294783302586, -274.0402769847039508 ) ) ;
#15341=CARTESIAN_POINT ( 'NONE',  ( -86.76039210456256967, -278.8940769487023772, -211.3228784931404221 ) ) ;
#15342=CARTESIAN_POINT ( 'NONE',  ( -11.18784957111032163, -272.7984835083657345, -201.2962092691876421 ) ) ;
#15343=CARTESIAN_POINT ( 'NONE',  ( -110.1944817108390282, -273.7391095985399261, -262.1942159385521336 ) ) ;
#15344=CARTESIAN_POINT ( 'NONE',  ( -46.21914874989020916, -274.8780235908361078, -197.6658681115683578 ) ) ;
#15345=CARTESIAN_POINT ( 'NONE',  ( -34.81320809752045875, -299.6834293582773512, -194.1604374374741724 ) ) ;
#15347=CARTESIAN_POINT ( 'NONE',  ( -7.255076896303360279, -274.6796336568085053, -339.4634301279916144 ) ) ;
#15348=CARTESIAN_POINT ( 'NONE',  ( -50.48139850148218244, -295.8758124243128691, -342.2724591918818078 ) ) ;
#15349=CARTESIAN_POINT ( 'NONE',  ( 4.133635785970411369, -293.0556478034519614, -331.1490397004779425 ) ) ;
#15351=CARTESIAN_POINT ( 'NONE',  ( -71.53786057731051073, -277.9841363965887240, -339.2824464234855100 ) ) ;
#15352=CARTESIAN_POINT ( 'NONE',  ( -38.08449000872437296, -274.2092686259905463, -197.3648970685308370 ) ) ;
#15353=CARTESIAN_POINT ( 'NONE',  ( -113.1133792082728462, -283.0990852358850134, -281.3165783458058513 ) ) ;
#15354=CARTESIAN_POINT ( 'NONE',  ( -110.1855073782314776, -298.3140285322057821, -288.9550740863743954 ) ) ;
#15356=CARTESIAN_POINT ( 'NONE',  ( -73.62685291481743377, -284.7545394330281852, -206.8171534796748858 ) ) ;
#15357=CARTESIAN_POINT ( 'NONE',  ( -110.9138627468296221, -276.6811061017833708, -278.8845582845285662 ) ) ;
#15358=CARTESIAN_POINT ( 'NONE',  ( -62.00426131226882376, -275.9537518484900147, -339.7487888401189480 ) ) ;
#15359=CARTESIAN_POINT ( 'NONE',  ( -44.77375041825170854, -285.1462579040637593, -345.0429320035668752 ) ) ;
#15360=CARTESIAN_POINT ( 'NONE',  ( -3.937601171315169957, -275.7079977478201727, -204.9918520094395262 ) ) ;
#15361=CARTESIAN_POINT ( 'NONE',  ( 37.16749025082013702, -273.7495129339185382, -254.3362449738000350 ) ) ;
#15362=CARTESIAN_POINT ( 'NONE',  ( -28.46734655870469055, -282.1645066135703246, -195.6678022783608242 ) ) ;
#15364=CARTESIAN_POINT ( 'NONE',  ( 27.45092162264288760, -288.9544822160695503, -231.3857146236530866 ) ) ;
#15366=CARTESIAN_POINT ( 'NONE',  ( 19.00382594025919403, -290.8640596368140905, -220.8427051785129720 ) ) ;
#15368=CARTESIAN_POINT ( 'NONE',  ( -75.40350267319112731, -296.3276379751258105, -207.5452894004086204 ) ) ;
#15369=CARTESIAN_POINT ( 'NONE',  ( -110.3986613925245450, -288.5208427580174657, -283.5347998072239193 ) ) ;
#15370=CARTESIAN_POINT ( 'NONE',  ( 139.3989977797154154, 177.7276089766264704, -238.0725708408485843 ) ) ;
#15372=CARTESIAN_POINT ( 'NONE',  ( -65.21199394003551220, -287.8895862575334945, -341.4518425499307455 ) ) ;
#15373=CARTESIAN_POINT ( 'NONE',  ( -3.233727128736103129, -284.1940206674063916, -335.8205728660128102 ) ) ;
#15374=CARTESIAN_POINT ( 'NONE',  ( -109.9509919666699034, -283.0791428576383737, -247.7818524211022577 ) ) ;
#15375=CARTESIAN_POINT ( 'NONE',  ( 8.172521695665620811, -283.8412485106957206, -328.2520732891190960 ) ) ;
#15376=CARTESIAN_POINT ( 'NONE',  ( -61.57859437390880686, -284.1779536486143343, -339.4447134093149998 ) ) ;
#15377=CARTESIAN_POINT ( 'NONE',  ( -95.99362198791807543, -291.8837106165035493, -317.6927569271431935 ) ) ;
#15378=CARTESIAN_POINT ( 'NONE',  ( -83.57078393854244780, -273.7710369225730460, -208.7426653384931967 ) ) ;
#15379=CARTESIAN_POINT ( 'NONE',  ( -7.511357110192556696, -286.7439872543364459, -339.7974549331641470 ) ) ;
#15380=CARTESIAN_POINT ( 'NONE',  ( 33.71354887436204706, -275.1733096831787293, -240.5560580419500809 ) ) ;
#15381=CARTESIAN_POINT ( 'NONE',  ( 34.71085874907662117, -295.7845293362111079, -289.9104346689396721 ) ) ;
#15383=CARTESIAN_POINT ( 'NONE',  ( -106.6379572354042296, -292.6233781216987495, -303.7686719486574702 ) ) ;
#15384=CARTESIAN_POINT ( 'NONE',  ( -21.29675257103413344, -281.5269861995448650, -342.1337916457709412 ) ) ;
#15385=CARTESIAN_POINT ( 'NONE',  ( -110.7008741339251259, -276.3420841252038826, -286.7458676169089813 ) ) ;
#15386=CARTESIAN_POINT ( 'NONE',  ( -52.38977702765697586, -272.3428288674879809, -195.4989944281992109 ) ) ;
#15387=CARTESIAN_POINT ( 'NONE',  ( 24.06551077319547005, -275.4501638977528728, -310.1160959191046800 ) ) ;
#15388=CARTESIAN_POINT ( 'NONE',  ( -55.19892289577111200, -293.3383958537947933, -198.8640736691187669 ) ) ;
#15389=CARTESIAN_POINT ( 'NONE',  ( 22.77424686552371824, -293.9120259033625757, -228.5122250550866738 ) ) ;
#15390=CARTESIAN_POINT ( 'NONE',  ( -109.0154977850382920, -286.5526682517989343, -251.8992452407488543 ) ) ;
#15391=CARTESIAN_POINT ( 'NONE',  ( 35.71823501086125674, -294.6942363690599223, -247.9813912079839326 ) ) ;
#15392=CARTESIAN_POINT ( 'NONE',  ( 36.62411581856360243, -295.1136947045292800, -289.9150522489528043 ) ) ;
#15393=CARTESIAN_POINT ( 'NONE',  ( -96.40966383013012830, -295.7849124579788054, -313.2773922716567085 ) ) ;
#15394=CARTESIAN_POINT ( 'NONE',  ( -61.88612845664857787, -291.3713609523749142, -341.2312222974078963 ) ) ;
#15395=CARTESIAN_POINT ( 'NONE',  ( -111.4908979686912858, -284.4587181892767944, -291.1191637506960888 ) ) ;
#15396=CARTESIAN_POINT ( 'NONE',  ( -108.9269296779008727, -271.0097198716212006, -245.5445833778888129 ) ) ;
#15397=CARTESIAN_POINT ( 'NONE',  ( -105.7851207363626003, -283.9294843761073253, -305.7549059128548379 ) ) ;
#15398=CARTESIAN_POINT ( 'NONE',  ( -111.5360518773532306, -280.4205367059468585, -279.0047666204628740 ) ) ;
#15399=CARTESIAN_POINT ( 'NONE',  ( -104.9574016360991919, -283.7297886563487168, -241.6780112830523137 ) ) ;
#15400=CARTESIAN_POINT ( 'NONE',  ( 32.98785508828261470, -285.2138356126249050, -244.3082043236840946 ) ) ;
#15401=CARTESIAN_POINT ( 'NONE',  ( -69.41752987730927771, -277.7742047141237549, -201.7069827068197014 ) ) ;
#15402=CARTESIAN_POINT ( 'NONE',  ( -35.93751134800100289, -122.5594593288581251, -363.2174194532766478 ) ) ;
#15404=CARTESIAN_POINT ( 'NONE',  ( -110.4520475260046481, -284.0526527651196034, -270.9035042900704866 ) ) ;
#15406=CARTESIAN_POINT ( 'NONE',  ( 23.09913496815175193, -283.3894092190927836, -317.4451948365138492 ) ) ;
#15407=CARTESIAN_POINT ( 'NONE',  ( -36.10269794830810497, -288.0957602359025600, -347.1288956867550155 ) ) ;
#15408=CARTESIAN_POINT ( 'NONE',  ( -95.52501399680663496, -279.4821460033404037, -319.5863559707076433 ) ) ;
#15409=CARTESIAN_POINT ( 'NONE',  ( -75.07828521310315750, -278.8592459885100538, -336.9137168734408760 ) ) ;
#15410=CARTESIAN_POINT ( 'NONE',  ( -19.53250049226435792, -280.1208348475300340, -199.5145310700542041 ) ) ;
#15411=CARTESIAN_POINT ( 'NONE',  ( -77.46921265032453618, -275.4907273521913567, -207.4196408772093037 ) ) ;
#15412=CARTESIAN_POINT ( 'NONE',  ( 28.10592367883777953, -294.0838060122432580, -311.0273911351308129 ) ) ;
#15413=CARTESIAN_POINT ( 'NONE',  ( -34.54098843903138061, -287.0370281848212244, -345.0040618070150344 ) ) ;
#15414=AXIS2_PLACEMENT_3D ( 'NONE', #44355, #8377, #45267 ) ;
#15415=CARTESIAN_POINT ( 'NONE',  ( -74.30881767538970450, -293.1691916583761781, -203.7287486985987925 ) ) ;
#15416=CARTESIAN_POINT ( 'NONE',  ( -68.66183837227877973, -294.3940262995200783, -336.6566932860676502 ) ) ;
#15417=CARTESIAN_POINT ( 'NONE',  ( -3.137608213132380364, -294.2538179820011237, -334.8759812553842607 ) ) ;
#15418=CARTESIAN_POINT ( 'NONE',  ( -112.0194285377326366, -291.8510213313587656, -252.9046180210496857 ) ) ;
#15419=CARTESIAN_POINT ( 'NONE',  ( 34.66606907960790807, -282.0375775403526291, -257.7605687045281115 ) ) ;
#15420=CARTESIAN_POINT ( 'NONE',  ( 53.14800697766726501, -298.0804408912529766, -193.6863325086212342 ) ) ;
#15421=CARTESIAN_POINT ( 'NONE',  ( -54.47082684962213506, -289.9179250305709274, -345.3817871544957825 ) ) ;
#15422=CARTESIAN_POINT ( 'NONE',  ( -8.530893964465663615, -280.8187867445068946, -340.4898669552225670 ) ) ;
#15424=CARTESIAN_POINT ( 'NONE',  ( 28.88771343880231512, -288.3967428443834820, -309.5964218560844188 ) ) ;
#15425=CARTESIAN_POINT ( 'NONE',  ( -89.68097257443268688, -285.6221978585015222, -219.3701080027280454 ) ) ;
#15427=CARTESIAN_POINT ( 'NONE',  ( 119.8541137665874032, 149.3386895696777685, -261.6380840896607083 ) ) ;
#15428=CARTESIAN_POINT ( 'NONE',  ( 184.3255359987551572, 260.6165026356828207, -150.9744038209046835 ) ) ;
#15429=CARTESIAN_POINT ( 'NONE',  ( -64.86740973677453326, -278.8803471481014640, -202.5751530804830054 ) ) ;
#15430=CARTESIAN_POINT ( 'NONE',  ( -108.4753526115228794, -277.2389246256303181, -288.1394287253564812 ) ) ;
#15431=CARTESIAN_POINT ( 'NONE',  ( 26.91524881597910834, -274.6613155780240163, -227.9725723138843421 ) ) ;
#15432=CARTESIAN_POINT ( 'NONE',  ( 169.0186518065400207, 229.7053051813165609, -190.5595449943317590 ) ) ;
#15434=CARTESIAN_POINT ( 'NONE',  ( -113.6215691676236190, -277.1832258824243240, -265.8903383180676201 ) ) ;
#15435=CARTESIAN_POINT ( 'NONE',  ( -4.117207549396958655, -280.6319489220272771, -337.2040674947708112 ) ) ;
#15436=CARTESIAN_POINT ( 'NONE',  ( 3.699105587511749338, -296.2685889135162824, -334.3732642774897954 ) ) ;
#15437=CARTESIAN_POINT ( 'NONE',  ( -12.24495194684063826, -292.8798780284144527, -201.6912972614359774 ) ) ;
#15438=CARTESIAN_POINT ( 'NONE',  ( -113.3132253104770513, -273.6360301137744386, -258.9914686285616199 ) ) ;
#15439=CARTESIAN_POINT ( 'NONE',  ( -15.72246093755871854, -287.4514675733697686, -340.6556792537484739 ) ) ;
#15440=CARTESIAN_POINT ( 'NONE',  ( -112.3457027523918725, -273.4159770912813769, -253.3990315088814782 ) ) ;
#15441=CARTESIAN_POINT ( 'NONE',  ( -99.89788960871300105, -297.2377200359368885, -232.6367136827935838 ) ) ;
#15444=CARTESIAN_POINT ( 'NONE',  ( -111.5859246497350910, -280.6521163567664416, -256.2522418109721229 ) ) ;
#15445=CARTESIAN_POINT ( 'NONE',  ( -49.20541722335731549, -280.9770700740090206, -198.0183347243558103 ) ) ;
#15446=CARTESIAN_POINT ( 'NONE',  ( -84.22333551785669670, -279.4466209132146446, -330.2283487039617285 ) ) ;
#15447=CARTESIAN_POINT ( 'NONE',  ( 9.944657221575299744, -273.1969317345193531, -213.7725295160784356 ) ) ;
#15450=CARTESIAN_POINT ( 'NONE',  ( -1.533896377987240323, -277.3924975820768850, -338.3461164124301490 ) ) ;
#15451=CARTESIAN_POINT ( 'NONE',  ( -7.350445041457863482, -278.6590430200135984, -339.1174624732529992 ) ) ;
#15452=CARTESIAN_POINT ( 'NONE',  ( -82.21502377928607075, -276.2259147438053333, -332.2076305431442051 ) ) ;
#15453=ORIENTED_EDGE ( 'NONE', *, *, #69844, .F. ) ;
#15455=CARTESIAN_POINT ( 'NONE',  ( 23.78809117464455980, -284.1292499200839075, -314.4461156251521743 ) ) ;
#15456=CARTESIAN_POINT ( 'NONE',  ( -14.78692970620623548, -291.5491870720394445, -200.7631003535099410 ) ) ;
#15457=CARTESIAN_POINT ( 'NONE',  ( -32.30480070587665864, -285.4626604036957929, -193.6150399180537818 ) ) ;
#15458=CARTESIAN_POINT ( 'NONE',  ( -109.9782385243363905, -282.6071293582365342, -284.5705270272298435 ) ) ;
#15459=CARTESIAN_POINT ( 'NONE',  ( -40.27587738680338703, -281.6644807898208001, -343.8918294037683268 ) ) ;
#15460=CARTESIAN_POINT ( 'NONE',  ( -59.87002246616999201, -280.9588795646532162, -200.4533483243079104 ) ) ;
#15461=CARTESIAN_POINT ( 'NONE',  ( -99.53540881432127208, -271.1200460983058633, -228.3527980389987988 ) ) ;
#15463=CARTESIAN_POINT ( 'NONE',  ( -91.87558171365287762, -282.2143529597015004, -323.5823184013495961 ) ) ;
#15464=CARTESIAN_POINT ( 'NONE',  ( -102.8434524688352667, -298.0648251110738443, -306.9983206699136531 ) ) ;
#15465=AXIS2_PLACEMENT_3D ( 'NONE', #2295, #37780, #30701 ) ;
#15466=CARTESIAN_POINT ( 'NONE',  ( -104.4823228387848957, -279.0998642985279616, -299.7378469757191510 ) ) ;
#15467=CARTESIAN_POINT ( 'NONE',  ( -112.0016947189301248, -286.6639379115852648, -261.6482749732219304 ) ) ;
#15468=VECTOR ( 'NONE', #3128, 1000.000000000000000 ) ;
#15470=CARTESIAN_POINT ( 'NONE',  ( -37.81109012966459915, -293.9664642839941848, -194.8025719700286231 ) ) ;
#15472=CARTESIAN_POINT ( 'NONE',  ( -0.5096664150300678209, -274.5628873235659171, -335.7528852756741458 ) ) ;
#15473=CARTESIAN_POINT ( 'NONE',  ( 21.35903660258810532, -287.4187249604672729, -319.9431946665179680 ) ) ;
#15474=CARTESIAN_POINT ( 'NONE',  ( -2.039019217071922796, -290.9276490029278079, -205.5381152348151375 ) ) ;
#15475=CARTESIAN_POINT ( 'NONE',  ( -70.69144971784091069, -276.1864441551169307, -335.8518629902656016 ) ) ;
#15476=CARTESIAN_POINT ( 'NONE',  ( -110.9580217513515663, -294.8208446344581830, -260.4080340269800899 ) ) ;
#15477=CARTESIAN_POINT ( 'NONE',  ( -12.10649988399451615, -293.7025721853072469, -201.2820442769315719 ) ) ;
#15480=CARTESIAN_POINT ( 'NONE',  ( -64.04188194062869854, -293.8740878990336114, -341.8440393241148740 ) ) ;
#15481=CARTESIAN_POINT ( 'NONE',  ( 19.26238690199036796, -288.4871869828853619, -222.9872636629539500 ) ) ;
#15482=CARTESIAN_POINT ( 'NONE',  ( -112.1398541117927579, -288.6214275298790994, -283.8216726500512550 ) ) ;
#15483=CARTESIAN_POINT ( 'NONE',  ( -18.30370430935523629, -290.2274056412199457, -341.4980935733968295 ) ) ;
#15485=CARTESIAN_POINT ( 'NONE',  ( -96.68361562349598159, -290.7578489211797432, -313.1529255233432423 ) ) ;
#15487=CARTESIAN_POINT ( 'NONE',  ( -84.90605288674601070, -290.8963931897126827, -330.4757758274485582 ) ) ;
#15488=CARTESIAN_POINT ( 'NONE',  ( -22.85709954863275328, -278.2565650340623051, -196.3580142372265414 ) ) ;
#15489=CARTESIAN_POINT ( 'NONE',  ( -75.00129581361970565, -279.8979010202619406, -203.2232066034774789 ) ) ;
#15490=CARTESIAN_POINT ( 'NONE',  ( -3.663025696490039618, -280.1511800364907572, -201.1260053622769419 ) ) ;
#15491=CARTESIAN_POINT ( 'NONE',  ( 20.21249047490515949, -284.8874804659265010, -222.2524768509212549 ) ) ;
#15493=CARTESIAN_POINT ( 'NONE',  ( -97.39115258327184677, -277.2924297602724550, -226.7156286179795188 ) ) ;
#15494=CARTESIAN_POINT ( 'NONE',  ( -14.06740595226352220, -280.7500629050644534, -341.6584382519707788 ) ) ;
#15495=CARTESIAN_POINT ( 'NONE',  ( -69.44095347752850955, -196.3684352495399423, -356.8806866962679010 ) ) ;
#15496=CARTESIAN_POINT ( 'NONE',  ( -86.34452415002552073, -277.8664675687668364, -211.7992629637615778 ) ) ;
#15497=CARTESIAN_POINT ( 'NONE',  ( -113.2952137877150705, -283.3345498565198000, -281.3459419085112359 ) ) ;
#15498=CARTESIAN_POINT ( 'NONE',  ( -91.24841961072959862, -274.0634702276702228, -220.8787716704212016 ) ) ;
#15499=CARTESIAN_POINT ( 'NONE',  ( -94.65661773434429449, -274.6668990126169660, -219.8278961034325221 ) ) ;
#15500=CARTESIAN_POINT ( 'NONE',  ( 30.29600990820854989, -275.5889779607466608, -298.0134113041055457 ) ) ;
#15501=CARTESIAN_POINT ( 'NONE',  ( -95.47709060472682552, -297.8992183653352299, -317.7656488081095745 ) ) ;
#15502=CARTESIAN_POINT ( 'NONE',  ( -5.624555881219731823, -288.8130865274976600, -340.5253735928897072 ) ) ;
#15503=CARTESIAN_POINT ( 'NONE',  ( 3.072819304755261438, -278.6697504338949329, -206.4558938566724748 ) ) ;
#15504=CARTESIAN_POINT ( 'NONE',  ( -74.67703883990867553, -291.4026685653622053, -203.0181711522665751 ) ) ;
#15505=CARTESIAN_POINT ( 'NONE',  ( -73.67207087498614726, -288.6058024108472182, -333.9641971604327750 ) ) ;
#15506=CARTESIAN_POINT ( 'NONE',  ( 37.65702769368315472, -291.5157384812855526, -267.5379728276618039 ) ) ;
#15509=CARTESIAN_POINT ( 'NONE',  ( -86.77562673980663988, -289.2693975491652623, -324.2282259305274010 ) ) ;
#15511=CARTESIAN_POINT ( 'NONE',  ( 11.91738437348854696, -287.6583459198519108, -211.4159385299737437 ) ) ;
#15512=CARTESIAN_POINT ( 'NONE',  ( 34.45848030099739390, -296.0519495502701943, -270.3284710469131937 ) ) ;
#15513=CARTESIAN_POINT ( 'NONE',  ( 15.30857153722725528, -293.3885980682417767, -326.2249623367883373 ) ) ;
#15514=CARTESIAN_POINT ( 'NONE',  ( -24.59912086932454756, -284.2081126969912930, -345.8531086079086094 ) ) ;
#15515=CARTESIAN_POINT ( 'NONE',  ( -107.7617144909671794, -284.1307738691438658, -289.6442625614449753 ) ) ;
#15516=CARTESIAN_POINT ( 'NONE',  ( 35.84662990274996019, -276.9549491958516114, -277.0478080881935625 ) ) ;
#15517=CARTESIAN_POINT ( 'NONE',  ( 36.46040943060042139, -291.7208780362105927, -281.8811912947693372 ) ) ;
#15518=CARTESIAN_POINT ( 'NONE',  ( -56.95302693766149105, -272.5885782481558408, -199.5795779481681222 ) ) ;
#15521=CARTESIAN_POINT ( 'NONE',  ( 38.04902157672568563, -293.4134731304052934, -285.9169327299435395 ) ) ;
#15522=CARTESIAN_POINT ( 'NONE',  ( -42.80371783198999225, -287.9028809908334665, -196.1088968441945610 ) ) ;
#15523=CARTESIAN_POINT ( 'NONE',  ( -111.3275404330224063, -297.8879251974468048, -249.9759473579094902 ) ) ;
#15524=CARTESIAN_POINT ( 'NONE',  ( 20.41609760707875409, -287.5732843027383296, -225.5511919691297180 ) ) ;
#15526=CARTESIAN_POINT ( 'NONE',  ( -113.0690263310504378, -277.4531231761198455, -282.9385692079628143 ) ) ;
#15527=CARTESIAN_POINT ( 'NONE',  ( -34.84962683864793576, -295.6730240235590941, -347.2187939663132283 ) ) ;
#15528=CARTESIAN_POINT ( 'NONE',  ( 17.73043949616242898, -286.4139552355005094, -322.3934628999368783 ) ) ;
#15529=CARTESIAN_POINT ( 'NONE',  ( 13.38508417406806750, -294.6986037307403876, -328.3328991369119194 ) ) ;
#15531=CARTESIAN_POINT ( 'NONE',  ( -98.31953436761223486, -291.4435006487648820, -230.0972434778849447 ) ) ;
#15535=CARTESIAN_POINT ( 'NONE',  ( 167.9831408986860311, 229.6749329237118502, -189.9962676830372459 ) ) ;
#15536=CARTESIAN_POINT ( 'NONE',  ( -26.73678813539466859, -287.7046817743762404, -194.7419480771833946 ) ) ;
#15537=CARTESIAN_POINT ( 'NONE',  ( -115.3288506153726871, -288.2666405000203440, -252.5284128619063608 ) ) ;
#15540=CARTESIAN_POINT ( 'NONE',  ( -40.99524215679190320, -279.3559304719699412, -193.5367140391501266 ) ) ;
#15541=CARTESIAN_POINT ( 'NONE',  ( 22.49070238628492291, -284.1681633019224478, -315.3279585992952434 ) ) ;
#15542=CARTESIAN_POINT ( 'NONE',  ( 199.0215121565617267, 282.8125914077994594, -111.1903278149338234 ) ) ;
#15543=CARTESIAN_POINT ( 'NONE',  ( -111.1472884868231148, -283.3787551812042693, -250.3800831854763942 ) ) ;
#15545=CARTESIAN_POINT ( 'NONE',  ( 33.68026516675332971, -285.9238120139998500, -292.8303560276534085 ) ) ;
#15546=CARTESIAN_POINT ( 'NONE',  ( -63.15882302151877781, -275.5798269534439555, -199.1306354260173350 ) ) ;
#15548=CARTESIAN_POINT ( 'NONE',  ( -96.15358268493778837, -297.6517714330614695, -226.9908198767547276 ) ) ;
#15549=CARTESIAN_POINT ( 'NONE',  ( -71.17261840074534973, -294.1932781082168731, -335.6186839874679890 ) ) ;
#15550=CARTESIAN_POINT ( 'NONE',  ( -72.78631088524953441, -278.1605068824746922, -338.6179612575067495 ) ) ;
#15551=CARTESIAN_POINT ( 'NONE',  ( 3.134106313982170988, -276.4915120258694401, -331.1123244962138870 ) ) ;
#15552=CARTESIAN_POINT ( 'NONE',  ( 29.67071477812140401, -276.1451962938810993, -232.9581353193223947 ) ) ;
#15553=CARTESIAN_POINT ( 'NONE',  ( -106.0744761891404693, -277.0321602773960876, -304.4997240623635548 ) ) ;
#15554=CARTESIAN_POINT ( 'NONE',  ( -108.0627147292225203, -262.2579186427535092, -317.5738021120087069 ) ) ;
#15555=CARTESIAN_POINT ( 'NONE',  ( 37.67789369394757415, -273.5799789553166192, -272.5411780619711521 ) ) ;
#15557=CARTESIAN_POINT ( 'NONE',  ( -100.2757451797973403, -298.5541765641321490, -227.0032316287117169 ) ) ;
#15560=CARTESIAN_POINT ( 'NONE',  ( -8.144417319489569707, -287.5234762706672313, -203.1171981764386203 ) ) ;
#15561=CARTESIAN_POINT ( 'NONE',  ( -94.55676660713815807, -285.6269370007227053, -320.3652196448921927 ) ) ;
#15562=CARTESIAN_POINT ( 'NONE',  ( 11.20794237688972927, -286.0941820544749703, -215.6412479039078107 ) ) ;
#15563=CARTESIAN_POINT ( 'NONE',  ( -102.5734509685682383, -276.4869920278521818, -304.8757394560932426 ) ) ;
#15564=CARTESIAN_POINT ( 'NONE',  ( -71.96432037833695006, -285.3754567050283413, -336.0280019457031244 ) ) ;
#15565=CARTESIAN_POINT ( 'NONE',  ( -30.17587885582971552, -278.6241839869974797, -196.9661724759061485 ) ) ;
#15566=CARTESIAN_POINT ( 'NONE',  ( 28.31344128722500741, -277.0735379453712994, -303.0889167322516755 ) ) ;
#15568=CARTESIAN_POINT ( 'NONE',  ( -67.08829714036308189, -274.1437299935051897, -203.6156482484107926 ) ) ;
#15569=CARTESIAN_POINT ( 'NONE',  ( -19.80303690281566986, -281.0747829459431841, -195.4963438305881596 ) ) ;
#15571=CARTESIAN_POINT ( 'NONE',  ( -10.71744063881215503, -283.2065319318710976, -342.6027311592188767 ) ) ;
#15575=CARTESIAN_POINT ( 'NONE',  ( 29.03776111825984074, -288.9305519403758922, -233.7273628332340252 ) ) ;
#15576=CARTESIAN_POINT ( 'NONE',  ( -109.0059822543751409, -289.5796578308784888, -243.4235014689797936 ) ) ;
#15577=CARTESIAN_POINT ( 'NONE',  ( -104.0881193809927652, -295.3451835055575430, -300.4435881306248461 ) ) ;
#15578=CARTESIAN_POINT ( 'NONE',  ( -27.85343086611573327, -291.5180707966947580, -193.9970591528559396 ) ) ;
#15579=CARTESIAN_POINT ( 'NONE',  ( 6.239210459243984985, -286.9286035570306694, -329.8503855643155589 ) ) ;
#15580=CARTESIAN_POINT ( 'NONE',  ( 0.3595220217773859583, -287.7711873389431503, -207.3276844743342906 ) ) ;
#15581=CARTESIAN_POINT ( 'NONE',  ( -69.91165696735023971, -294.1233781216987495, -202.8022627189028810 ) ) ;
#15582=CARTESIAN_POINT ( 'NONE',  ( 36.70468566338232819, -289.7094520672786757, -282.5994867599419536 ) ) ;
#15583=CARTESIAN_POINT ( 'NONE',  ( -102.2289997878032040, -288.0449517667890404, -308.4070688725983587 ) ) ;
#15584=CARTESIAN_POINT ( 'NONE',  ( -71.50806339830540992, -284.4564413394722919, -335.1381823614480027 ) ) ;
#15585=CARTESIAN_POINT ( 'NONE',  ( -110.7688462590590603, -292.3463345877702864, -286.4385133592856505 ) ) ;
#15586=CARTESIAN_POINT ( 'NONE',  ( 82.15764098272329363, -298.8646310024031436, -193.4766962576139804 ) ) ;
#15587=DIRECTION ( 'NONE',  ( 0.000000000000000000, 0.000000000000000000, 1.000000000000000000 ) ) ;
#15588=CARTESIAN_POINT ( 'NONE',  ( -34.84395483231872248, -300.0033357693390030, -194.8003003694630308 ) ) ;
#15589=CARTESIAN_POINT ( 'NONE',  ( 25.27978124254390480, -280.2285769419000303, -232.4323528950670834 ) ) ;
#15590=CARTESIAN_POINT ( 'NONE',  ( -95.86110629276807060, -281.9066092695691168, -317.2908288172852735 ) ) ;
#15591=CARTESIAN_POINT ( 'NONE',  ( -22.13951346636238071, -294.0593382188949931, -345.6807856710722149 ) ) ;
#15592=CARTESIAN_POINT ( 'NONE',  ( -72.36776059174798092, -271.8222390082464699, -205.1031827726991992 ) ) ;
#15593=CARTESIAN_POINT ( 'NONE',  ( -6.941515913247738645, -274.7299029188646955, -338.3106801618453119 ) ) ;
#15594=CARTESIAN_POINT ( 'NONE',  ( -107.1806343046838066, -298.1709387182804676, -247.3137143412378691 ) ) ;
#15595=FACE_OUTER_BOUND ( 'NONE', #73538, .T. ) ;
#15596=CARTESIAN_POINT ( 'NONE',  ( -108.4966480947757930, -294.4485538557960354, -297.1732855322821365 ) ) ;
#15598=CARTESIAN_POINT ( 'NONE',  ( -10.25637852233398917, -296.1168338599671301, -338.7845077774825313 ) ) ;
#15600=CARTESIAN_POINT ( 'NONE',  ( -36.98451421717186349, -295.8503687901634294, -343.5341749740960040 ) ) ;
#15603=CARTESIAN_POINT ( 'NONE',  ( -101.1128170511424571, -283.1094614313733473, -230.2157390696378627 ) ) ;
#15604=CARTESIAN_POINT ( 'NONE',  ( -106.8692721386701265, -296.2551786450661666, -292.7714844526203706 ) ) ;
#15606=CARTESIAN_POINT ( 'NONE',  ( -109.9772555785848880, -284.8745343175664857, -244.8057646412964630 ) ) ;
#15607=CARTESIAN_POINT ( 'NONE',  ( 36.15354970941837820, -283.6965394059326400, -287.9595439960593808 ) ) ;
#15608=CARTESIAN_POINT ( 'NONE',  ( 35.05113572283053003, -287.5512505406355217, -296.6890974025344576 ) ) ;
#15609=CARTESIAN_POINT ( 'NONE',  ( -52.72230746304008164, -289.8546012352798584, -197.0722341398119681 ) ) ;
#15610=CARTESIAN_POINT ( 'NONE',  ( -112.3867484786949404, -277.6906130078346564, -287.1406741517341175 ) ) ;
#15611=CARTESIAN_POINT ( 'NONE',  ( -106.6379572354042153, -276.4809262143061233, -236.9535640164627068 ) ) ;
#15614=CARTESIAN_POINT ( 'NONE',  ( -8.082631778666776512, -285.2390984480305747, -203.0481368793026604 ) ) ;
#15615=CARTESIAN_POINT ( 'NONE',  ( -108.5167148168941225, -289.1085914890034019, -298.9200008927197700 ) ) ;
#15617=CARTESIAN_POINT ( 'NONE',  ( -75.02965664345900620, -278.9693264961290993, -336.8308421195906135 ) ) ;
#15618=CARTESIAN_POINT ( 'NONE',  ( -3.980152954366232620, -292.6345629494124978, -337.9432552927411280 ) ) ;
#15619=CARTESIAN_POINT ( 'NONE',  ( 15.27756267139046820, -280.4873756404109031, -219.6598301418038943 ) ) ;
#15620=CARTESIAN_POINT ( 'NONE',  ( -34.85251716959677282, -295.1883692188969803, -347.3208735222163455 ) ) ;
#15621=CONICAL_SURFACE ( 'NONE', #82114, 2.738891987356051327, 0.09862129276975473147 ) ;
#15622=CARTESIAN_POINT ( 'NONE',  ( -26.79740472569955045, -284.2649598192937219, -195.4879523725978174 ) ) ;
#15623=CARTESIAN_POINT ( 'NONE',  ( -111.7366965054040264, -280.6794707973262462, -260.4578789101729512 ) ) ;
#15624=CARTESIAN_POINT ( 'NONE',  ( -31.59581466333957067, -294.0367225890842633, -343.4209350127624134 ) ) ;
#15628=CARTESIAN_POINT ( 'NONE',  ( 19.19416639992928353, -282.8529442103424572, -221.6019670233719125 ) ) ;
#15629=CARTESIAN_POINT ( 'NONE',  ( -106.7632923745864417, -296.3637089674620029, -247.4273004536887584 ) ) ;
#15631=CARTESIAN_POINT ( 'NONE',  ( -85.28047601435909542, -270.9094976428775681, -210.1954327657594206 ) ) ;
#15632=CARTESIAN_POINT ( 'NONE',  ( -67.46290370518146062, -272.8641379301053576, -199.6725622195420726 ) ) ;
#15633=CARTESIAN_POINT ( 'NONE',  ( -108.1079520002728600, -290.6225939575098209, -252.3899727515743336 ) ) ;
#15634=CARTESIAN_POINT ( 'NONE',  ( -108.2910374738124517, -280.3336870025995609, -250.3919718224957762 ) ) ;
#15635=CARTESIAN_POINT ( 'NONE',  ( -29.92956130563193184, -275.7476633421790666, -196.9342794773952505 ) ) ;
#15636=CARTESIAN_POINT ( 'NONE',  ( -16.34253484235405551, -284.3854089957309839, -343.6652401631999965 ) ) ;
#15637=CARTESIAN_POINT ( 'NONE',  ( 18.78815316669153290, -281.0154728718585488, -317.6730118753061447 ) ) ;
#15638=CARTESIAN_POINT ( 'NONE',  ( -0.4652335564866330597, -278.5625625254471629, -335.7278345602061904 ) ) ;
#15640=CARTESIAN_POINT ( 'NONE',  ( -60.86910050608528877, -273.5885139934989638, -196.9879500593584680 ) ) ;
#15641=CARTESIAN_POINT ( 'NONE',  ( -82.62401545215251986, -293.3485412286007090, -211.2126606203711958 ) ) ;
#15645=CARTESIAN_POINT ( 'NONE',  ( 35.89638832292738613, -291.9386181222029677, -289.7644136533795631 ) ) ;
#15646=CARTESIAN_POINT ( 'NONE',  ( -31.32840057402644263, -273.6377638889694595, -197.5348005380731706 ) ) ;
#15648=CARTESIAN_POINT ( 'NONE',  ( -36.40648853187516920, -293.5837930312608819, -194.0472653596006012 ) ) ;
#15649=CARTESIAN_POINT ( 'NONE',  ( -95.95921662488163406, -286.4090924074130839, -317.1477375740089997 ) ) ;
#15650=CARTESIAN_POINT ( 'NONE',  ( 1.485532896573637407, -293.7636489305879195, -204.2667656040680413 ) ) ;
#15651=CARTESIAN_POINT ( 'NONE',  ( 34.78978824073960396, -289.2954485892807952, -250.4343316301820153 ) ) ;
#15652=CARTESIAN_POINT ( 'NONE',  ( 37.43247904811050120, -273.6044406496577039, -274.4372635320963809 ) ) ;
#15653=CARTESIAN_POINT ( 'NONE',  ( -51.53190311712203453, -279.1552107154237774, -343.4360954657726097 ) ) ;
#15654=CARTESIAN_POINT ( 'NONE',  ( 36.63516107616717221, -291.7450886635492679, -279.1034642373022621 ) ) ;
#15655=CARTESIAN_POINT ( 'NONE',  ( -86.02939095455678853, -281.2464614706670432, -212.2426167304207354 ) ) ;
#15657=CARTESIAN_POINT ( 'NONE',  ( -4.821557711363796628, -282.2782934457702027, -335.7409912163431045 ) ) ;
#15658=CARTESIAN_POINT ( 'NONE',  ( -98.33889595381744186, -280.2542030202112073, -223.8549429124280721 ) ) ;
#15659=CIRCLE ( 'NONE', #80675, 5.343514653206204557 ) ;
#15660=CARTESIAN_POINT ( 'NONE',  ( -55.62236848749311946, -282.0773174121798661, -344.7508073339952261 ) ) ;
#15661=CARTESIAN_POINT ( 'NONE',  ( 18.73952676063448308, -277.2105001825364639, -322.7797807240210659 ) ) ;
#15664=CARTESIAN_POINT ( 'NONE',  ( 32.39405704835434108, -277.4712245351720412, -301.3390443492152713 ) ) ;
#15665=CARTESIAN_POINT ( 'NONE',  ( -6.941161984400275209, -285.1233781216987495, -333.4151289067050357 ) ) ;
#15668=CARTESIAN_POINT ( 'NONE',  ( -33.71597685990347060, -300.0976955582013943, -195.3598731451911021 ) ) ;
#15670=CARTESIAN_POINT ( 'NONE',  ( -95.36745559087739821, -292.2599202865949906, -225.5589106980830536 ) ) ;
#15671=CARTESIAN_POINT ( 'NONE',  ( -40.60229248747013031, -275.1134375053601957, -344.9474195032431112 ) ) ;
#15672=CARTESIAN_POINT ( 'NONE',  ( -67.62910702470186664, -291.2042600439678495, -340.0507657006041313 ) ) ;
#15673=CARTESIAN_POINT ( 'NONE',  ( -46.99973260817423437, -291.2748188540548426, -197.8999899439994579 ) ) ;
#15674=CARTESIAN_POINT ( 'NONE',  ( 37.76350133194356573, -287.2695260824559114, -287.1166195608068961 ) ) ;
#15676=CARTESIAN_POINT ( 'NONE',  ( 35.72886334755724391, -291.8441518527105245, -248.0161175045146251 ) ) ;
#15677=CARTESIAN_POINT ( 'NONE',  ( -109.7684933844223281, -282.7671163252316546, -284.5315109020893942 ) ) ;
#15678=CARTESIAN_POINT ( 'NONE',  ( -78.84570555296532746, -291.4780574855929558, -331.9720196402687975 ) ) ;
#15679=CARTESIAN_POINT ( 'NONE',  ( -105.2287869595842977, -283.4147931306565624, -241.5586038003118006 ) ) ;
#15680=CARTESIAN_POINT ( 'NONE',  ( -1.741765096175014627, -281.8496173591730667, -206.0657985231597991 ) ) ;
#15681=CARTESIAN_POINT ( 'NONE',  ( -80.39869404468016967, -290.5609782341948630, -333.9777894127583977 ) ) ;
#15683=CARTESIAN_POINT ( 'NONE',  ( -39.70950334026598227, -280.5139987854534525, -197.3254273463019501 ) ) ;
#15684=CARTESIAN_POINT ( 'NONE',  ( -16.71868838367480592, -291.1077458807506559, -196.5864603815265639 ) ) ;
#15685=CARTESIAN_POINT ( 'NONE',  ( 38.12965419157688984, -288.1741310256004454, -255.9308200620623666 ) ) ;
#15686=CARTESIAN_POINT ( 'NONE',  ( 30.31156959021290831, -288.5201206140747558, -307.1135440825466389 ) ) ;
#15687=CARTESIAN_POINT ( 'NONE',  ( -79.31101823185777278, -285.6348940655125261, -210.5698675560418280 ) ) ;
#15688=ORIENTED_EDGE ( 'NONE', *, *, #51345, .T. ) ;
#15690=CARTESIAN_POINT ( 'NONE',  ( 36.58402615480707709, -295.6241951317577445, -287.0116963799118821 ) ) ;
#15692=CARTESIAN_POINT ( 'NONE',  ( -93.34000908395449869, -294.5216563131037333, -322.5099454494621227 ) ) ;
#15693=AXIS2_PLACEMENT_3D ( 'NONE', #73314, #38223, #88426 ) ;
#15695=CARTESIAN_POINT ( 'NONE',  ( -32.41667044919245200, -276.0474209155116796, -343.4807504083718186 ) ) ;
#15696=CARTESIAN_POINT ( 'NONE',  ( -99.00572534570937933, -296.5128873753518519, -224.3950392202188482 ) ) ;
#15697=CARTESIAN_POINT ( 'NONE',  ( 36.31492657235076393, -292.0016308222263319, -268.0353721416071835 ) ) ;
#15698=CARTESIAN_POINT ( 'NONE',  ( -75.71714431431529135, -295.7726619851313785, -207.0142731760786035 ) ) ;
#15699=CARTESIAN_POINT ( 'NONE',  ( 34.45920473183720389, -294.9577614113862865, -285.6451458672650006 ) ) ;
#15700=CARTESIAN_POINT ( 'NONE',  ( 34.07968623757008686, -294.8496097595959782, -286.9455817794044492 ) ) ;
#15703=CARTESIAN_POINT ( 'NONE',  ( 14.20255407332929387, -292.3298601340402456, -325.0714303866116097 ) ) ;
#15704=CARTESIAN_POINT ( 'NONE',  ( -37.81818092046705715, -300.0463442340226266, -195.3612717124876497 ) ) ;
#15705=CARTESIAN_POINT ( 'NONE',  ( -71.27115696686891511, -290.4528696796340341, -335.2767519414826438 ) ) ;
#15706=CARTESIAN_POINT ( 'NONE',  ( -23.51067229161319716, -295.2038797835400601, -342.1120413905046007 ) ) ;
#15707=CARTESIAN_POINT ( 'NONE',  ( -76.92890028663416047, -279.5590586656325058, -334.5408551758219460 ) ) ;
#15708=CARTESIAN_POINT ( 'NONE',  ( -42.38074216411054351, -278.6746807049123618, -194.0203927541775784 ) ) ;
#15710=CARTESIAN_POINT ( 'NONE',  ( -107.9805766389407324, -272.2898811240633563, -239.8379718082779277 ) ) ;
#15711=CARTESIAN_POINT ( 'NONE',  ( 32.42836794541195644, -279.2908425936963681, -244.2621535599756726 ) ) ;
#15712=CARTESIAN_POINT ( 'NONE',  ( -110.9528672262496087, -277.2017763639781833, -250.6172295769206073 ) ) ;
#15713=CARTESIAN_POINT ( 'NONE',  ( -100.3404162136024951, -277.1047367088375495, -229.2646613154101090 ) ) ;
#15714=CARTESIAN_POINT ( 'NONE',  ( -94.82665083913092019, -295.8793068962090729, -224.5711199316950513 ) ) ;
#15715=CARTESIAN_POINT ( 'NONE',  ( -92.90992337966571313, -275.2550195736002934, -219.9719367496673783 ) ) ;
#15718=CARTESIAN_POINT ( 'NONE',  ( -111.5187946762251698, -288.4017120755921724, -283.7068696385525755 ) ) ;
#15719=CARTESIAN_POINT ( 'NONE',  ( -111.5419714876580741, -290.2943815622888337, -290.9358532218086566 ) ) ;
#15720=CARTESIAN_POINT ( 'NONE',  ( 18.65270835133079785, -276.8548607424910415, -220.1383267602795968 ) ) ;
#15721=CARTESIAN_POINT ( 'NONE',  ( -107.2720668098868941, -270.9062053259660843, -243.1118168049154633 ) ) ;
#15722=CARTESIAN_POINT ( 'NONE',  ( -60.45159488267000825, -284.9571876438917570, -197.0247525413947187 ) ) ;
#15724=CARTESIAN_POINT ( 'NONE',  ( -22.84022592749805369, -280.8665639038884478, -343.9980578094197767 ) ) ;
#15726=CARTESIAN_POINT ( 'NONE',  ( -32.11376847893124165, -290.9144513123974889, -197.1377792708069592 ) ) ;
#15727=CARTESIAN_POINT ( 'NONE',  ( -104.5946170076872619, -283.1105473254152116, -238.8082966797575750 ) ) ;
#15730=CARTESIAN_POINT ( 'NONE',  ( 37.41599315172956608, -291.6293351546223107, -276.3850653720522814 ) ) ;
#15731=CARTESIAN_POINT ( 'NONE',  ( -108.9433452175861987, -279.9182908714823839, -288.2917687642296869 ) ) ;
#15732=CARTESIAN_POINT ( 'NONE',  ( -88.04715580857174473, -284.9478374354295056, -327.8511397666733274 ) ) ;
#15733=CARTESIAN_POINT ( 'NONE',  ( 20.75956128145462998, -272.9699373103212565, -222.0542072548558110 ) ) ;
#15734=CARTESIAN_POINT ( 'NONE',  ( -102.2383922971621359, -285.0065767237442742, -236.9332950574640790 ) ) ;
#15735=CARTESIAN_POINT ( 'NONE',  ( -16.19431822141394406, -278.1987515482655908, -340.8997570737070077 ) ) ;
#15736=CARTESIAN_POINT ( 'NONE',  ( -70.51690510617177665, -278.3041081003494810, -335.5685370552156996 ) ) ;
#15738=CARTESIAN_POINT ( 'NONE',  ( -99.74064001227507958, -285.9889349028352399, -312.0640274430530212 ) ) ;
#15743=CARTESIAN_POINT ( 'NONE',  ( -90.71360426056845938, -295.6168412863164576, -325.9362385528231698 ) ) ;
#15744=CARTESIAN_POINT ( 'NONE',  ( 0.9921854987479219457, -288.5458788378502391, -206.2512012368181047 ) ) ;
#15746=CARTESIAN_POINT ( 'NONE',  ( -88.47809603358389552, -294.9094976428775681, -206.1857440867352693 ) ) ;
#15747=CARTESIAN_POINT ( 'NONE',  ( -95.66175755329258834, -278.1471443202430578, -220.5387092342852213 ) ) ;
#15748=CARTESIAN_POINT ( 'NONE',  ( -41.98464699157413804, -290.3944247489505983, -194.3026966182522415 ) ) ;
#15749=VECTOR ( 'NONE', #16529, 1000.000000000000000 ) ;
#15750=CARTESIAN_POINT ( 'NONE',  ( -111.0110390225973873, -286.0288001858123721, -273.6885650728635255 ) ) ;
#15751=CARTESIAN_POINT ( 'NONE',  ( -49.32778712253682585, -281.6574303330163502, -197.3247727152945572 ) ) ;
#15752=CARTESIAN_POINT ( 'NONE',  ( 23.38204111116941064, -288.3540016237112695, -223.9582792730560072 ) ) ;
#15753=CARTESIAN_POINT ( 'NONE',  ( 37.51450298795468541, -283.4927118020830790, -265.7189739419508214 ) ) ;
#15754=CARTESIAN_POINT ( 'NONE',  ( -84.86471090653175509, -277.8534161338482704, -331.0140421337385419 ) ) ;
#15755=CARTESIAN_POINT ( 'NONE',  ( -103.6432370432231664, -271.0139915167394520, -235.5483136870002454 ) ) ;
#15756=CARTESIAN_POINT ( 'NONE',  ( -45.27125990234764430, -279.7877971359382627, -193.7175141029504744 ) ) ;
#15757=AXIS2_PLACEMENT_3D ( 'NONE', #58704, #44003, #72900 ) ;
#15758=CARTESIAN_POINT ( 'NONE',  ( -32.63600604481754175, -275.9724781262844999, -196.2624705463541659 ) ) ;
#15761=CARTESIAN_POINT ( 'NONE',  ( -54.42813229853333468, -285.7662352645560873, -345.3683826091709648 ) ) ;
#15762=CARTESIAN_POINT ( 'NONE',  ( -67.11763380038603088, -271.9069839684858607, -200.4514062885034207 ) ) ;
#15764=CARTESIAN_POINT ( 'NONE',  ( -59.74654628216803331, -279.2617300106088578, -200.7663338298953875 ) ) ;
#15765=CIRCLE ( 'NONE', #91372, 6.654241149514406040 ) ;
#15766=CARTESIAN_POINT ( 'NONE',  ( 0.8623889957438575227, -277.7597621792862697, -336.8174971393888200 ) ) ;
#15767=CARTESIAN_POINT ( 'NONE',  ( -35.91562233682809335, -282.0934631412376348, -347.1256543763460627 ) ) ;
#15768=CARTESIAN_POINT ( 'NONE',  ( -23.57500759919864564, -290.6340851210343317, -343.1352824096118184 ) ) ;
#15769=CARTESIAN_POINT ( 'NONE',  ( -36.56901364325128867, -299.5817749106086012, -194.0542508093429035 ) ) ;
#15770=CARTESIAN_POINT ( 'NONE',  ( -34.79137658881326445, -299.2884837342763831, -193.7576786726185674 ) ) ;
#15771=CARTESIAN_POINT ( 'NONE',  ( 37.03190257185073619, -295.6647713112477618, -279.0999586585848533 ) ) ;
#15772=CARTESIAN_POINT ( 'NONE',  ( 37.18050840112420730, -279.4572050373725460, -262.9956068851622604 ) ) ;
#15773=CARTESIAN_POINT ( 'NONE',  ( -62.56224024776824422, -271.7424425916609607, -200.1060743341718933 ) ) ;
#15774=CARTESIAN_POINT ( 'NONE',  ( -112.6994222293774897, -286.2994677473962497, -258.7141483890073914 ) ) ;
#15776=CARTESIAN_POINT ( 'NONE',  ( -58.79265596617397449, -288.2564142794927307, -340.5146667550876600 ) ) ;
#15777=CARTESIAN_POINT ( 'NONE',  ( -94.25799649422008031, -240.8346478425894759, -341.8059174816269206 ) ) ;
#15779=CARTESIAN_POINT ( 'NONE',  ( 31.15113858071259401, -286.5668891689415432, -304.3527590392434945 ) ) ;
#15780=CARTESIAN_POINT ( 'NONE',  ( -34.58145317239293348, -288.6833730786188426, -343.3796701595642276 ) ) ;
#15782=CARTESIAN_POINT ( 'NONE',  ( -87.55796226229870172, -286.4503291221897712, -212.3268524840556211 ) ) ;
#15783=CARTESIAN_POINT ( 'NONE',  ( -59.19728555027650430, -277.6762602717579966, -340.0347921541303435 ) ) ;
#15784=CARTESIAN_POINT ( 'NONE',  ( 27.79710632349152633, -291.9397314209022056, -229.7832409918204348 ) ) ;
#15785=CARTESIAN_POINT ( 'NONE',  ( 13.61945179376667880, -283.0119442179482689, -328.0191005904653139 ) ) ;
#15786=CARTESIAN_POINT ( 'NONE',  ( 25.37164984025568870, -283.6519863530356247, -313.8552863653348481 ) ) ;
#15787=CARTESIAN_POINT ( 'NONE',  ( -93.41322580413236665, -284.1651751784793873, -323.1225336249639213 ) ) ;
#15788=CARTESIAN_POINT ( 'NONE',  ( -19.53350555847921655, -280.6207156214569522, -199.4924618051631455 ) ) ;
#15789=CARTESIAN_POINT ( 'NONE',  ( 21.31550574532286291, -272.4094976428775681, -223.6242672951989618 ) ) ;
#15790=CARTESIAN_POINT ( 'NONE',  ( -55.96988853928130681, -169.5567205125497026, -364.5607778869738809 ) ) ;
#15792=CARTESIAN_POINT ( 'NONE',  ( -37.79595051760566093, -279.0579763670951934, -345.2058430138453105 ) ) ;
#15793=CARTESIAN_POINT ( 'NONE',  ( 63.86165590144513260, 48.22071679732245997, -318.3204609132440055 ) ) ;
#15794=CARTESIAN_POINT ( 'NONE',  ( -31.96053399027169561, -124.1536744858074144, -360.9188437396628615 ) ) ;
#15795=CARTESIAN_POINT ( 'NONE',  ( -108.8771599182628762, -296.0998013240203477, -255.2486996240658641 ) ) ;
#15796=CARTESIAN_POINT ( 'NONE',  ( 23.11941843600870428, -293.6968422706145816, -317.9635528164654374 ) ) ;
#15797=CARTESIAN_POINT ( 'NONE',  ( -11.69923036777068504, -92.83970553864392627, -356.5485982400477383 ) ) ;
#15798=CARTESIAN_POINT ( 'NONE',  ( -91.20719530715918211, -295.8791242684621920, -216.1659639444002039 ) ) ;
#15799=CARTESIAN_POINT ( 'NONE',  ( -103.5722528561838800, -288.5156620334610693, -302.9180573094117221 ) ) ;
#15800=CARTESIAN_POINT ( 'NONE',  ( -38.33545915039621121, -296.9251556898597642, -344.5896699455098542 ) ) ;
#15801=CARTESIAN_POINT ( 'NONE',  ( 27.47323519179343876, -289.3376964818619967, -305.1143548479905121 ) ) ;
#15803=CARTESIAN_POINT ( 'NONE',  ( -3.322242422785143923, -295.5552343417230645, -339.1906236281188285 ) ) ;
#15804=CARTESIAN_POINT ( 'NONE',  ( 23.58191507446265334, -287.4843554956995035, -229.9421043074399051 ) ) ;
#15805=CARTESIAN_POINT ( 'NONE',  ( -65.38228815324573873, -296.4886999787862010, -199.0181447060146525 ) ) ;
#15806=CARTESIAN_POINT ( 'NONE',  ( 13.16463340631999479, -293.5402353310277022, -212.4536996931710746 ) ) ;
#15808=CARTESIAN_POINT ( 'NONE',  ( 23.12720196275153484, -294.6813772648756640, -317.9536647553479156 ) ) ;
#15809=CARTESIAN_POINT ( 'NONE',  ( -108.4279585600876601, -290.9386064109465906, -253.7010609757184909 ) ) ;
#15812=CARTESIAN_POINT ( 'NONE',  ( -0.7643527836910239959, -276.4541324976058831, -204.2297539535574629 ) ) ;
#15813=CARTESIAN_POINT ( 'NONE',  ( 28.17096716750732810, -273.8250393617002487, -230.5595654155608258 ) ) ;
#15816=CARTESIAN_POINT ( 'NONE',  ( 5.831565484502884367, -275.9914444384368721, -334.0446797504306460 ) ) ;
#15817=CARTESIAN_POINT ( 'NONE',  ( -62.28108434329747922, -272.1221451649846017, -200.9027309463273809 ) ) ;
#15818=CARTESIAN_POINT ( 'NONE',  ( 34.43045383032324480, -273.9379818480910558, -289.3248570320944850 ) ) ;
#15819=CARTESIAN_POINT ( 'NONE',  ( -65.94638528093550178, -274.7485101320852436, -202.8629842196025947 ) ) ;
#15820=CARTESIAN_POINT ( 'NONE',  ( -74.40277007354357863, -274.4878848261452049, -207.1368270804752569 ) ) ;
#15821=CARTESIAN_POINT ( 'NONE',  ( -36.57141465482660436, -299.6617648581236040, -194.1609068640118494 ) ) ;
#15822=CARTESIAN_POINT ( 'NONE',  ( -3.278009125179975669, -272.5197785983277754, -203.1301239395667437 ) ) ;
#15823=CARTESIAN_POINT ( 'NONE',  ( -36.98673327514982390, -295.6989739534406567, -343.4746312403531192 ) ) ;
#15824=CARTESIAN_POINT ( 'NONE',  ( -34.29482001438502436, -293.5878205805398693, -343.8872455823365044 ) ) ;
#15825=DIRECTION ( 'NONE',  ( -1.000000000000000000, -0.000000000000000000, -0.000000000000000000 ) ) ;
#15826=CARTESIAN_POINT ( 'NONE',  ( -35.70652650738632161, -277.5245315989930077, -347.2953146444539811 ) ) ;
#15827=CARTESIAN_POINT ( 'NONE',  ( 33.50866773477660843, -275.4867835498943691, -252.7763126600675605 ) ) ;
#15828=CARTESIAN_POINT ( 'NONE',  ( -108.8480569770757285, -282.8887269668780959, -297.7143281265255155 ) ) ;
#15829=CARTESIAN_POINT ( 'NONE',  ( -89.42299444709324518, -297.7833327765368949, -324.6320819047000441 ) ) ;
#15831=CARTESIAN_POINT ( 'NONE',  ( -77.12832246288606086, -284.7013812388969427, -208.9037307011588211 ) ) ;
#15833=CARTESIAN_POINT ( 'NONE',  ( -108.8044456165321776, -276.5410567607178223, -289.6237767427979293 ) ) ;
#15834=CARTESIAN_POINT ( 'NONE',  ( -59.38867912442427865, -275.9179900232000477, -340.5701318852129020 ) ) ;
#15835=CARTESIAN_POINT ( 'NONE',  ( 19.46028180675816799, -284.2314646432311065, -319.3552285864406599 ) ) ;
#15836=CARTESIAN_POINT ( 'NONE',  ( -19.18817475961845886, -275.4959466997436266, -199.1917435567324333 ) ) ;
#15838=CARTESIAN_POINT ( 'NONE',  ( 21.10378306268967208, -274.6169536895415604, -319.2545317751090010 ) ) ;
#15839=CARTESIAN_POINT ( 'NONE',  ( -20.19967638916713426, -282.2719182001559375, -197.1217323681618439 ) ) ;
#15841=CARTESIAN_POINT ( 'NONE',  ( 0.7737664981769470929, -288.4764068715076064, -205.1040166087259990 ) ) ;
#15842=CARTESIAN_POINT ( 'NONE',  ( -100.2168347810491724, -289.1043477193641138, -229.3815903185768832 ) ) ;
#15845=CARTESIAN_POINT ( 'NONE',  ( -101.1375842259761981, -271.7348080440483500, -233.7714437810683421 ) ) ;
#15846=CARTESIAN_POINT ( 'NONE',  ( -108.9231018478902939, -288.4339240464086060, -290.2222898316994701 ) ) ;
#15847=CARTESIAN_POINT ( 'NONE',  ( 197.9739649220119588, 291.4634315377682583, -67.91333382494548232 ) ) ;
#15849=CARTESIAN_POINT ( 'NONE',  ( 0.3597301801255887166, -287.0396685991814252, -336.7631898778850541 ) ) ;
#15850=CARTESIAN_POINT ( 'NONE',  ( -57.46570152981070834, -284.0358730944445824, -197.0330485416895385 ) ) ;
#15851=CARTESIAN_POINT ( 'NONE',  ( -83.82903660226966736, -291.3927718394438102, -214.0767724899135374 ) ) ;
#15852=CARTESIAN_POINT ( 'NONE',  ( 35.93731676802683950, -282.8820859717162080, -263.0751017122723283 ) ) ;
#15853=CARTESIAN_POINT ( 'NONE',  ( 17.73314211791389994, -283.0405946407308875, -318.5208883191551195 ) ) ;
#15854=CARTESIAN_POINT ( 'NONE',  ( -59.51863613430510469, -291.3178376571415242, -342.3791039995995220 ) ) ;
#15855=CARTESIAN_POINT ( 'NONE',  ( -99.55247379169004773, -273.4883377789485053, -224.9343960973226046 ) ) ;
#15856=CARTESIAN_POINT ( 'NONE',  ( -48.67756867471482707, -287.2751222521179670, -345.1188901777998126 ) ) ;
#15857=CARTESIAN_POINT ( 'NONE',  ( 11.78569239055504880, -274.7124983179081141, -211.0001866675216888 ) ) ;
#15858=CARTESIAN_POINT ( 'NONE',  ( -52.73300147527349679, -293.8340134860398507, -197.2672699442896658 ) ) ;
#15860=CARTESIAN_POINT ( 'NONE',  ( -85.28047601435908120, -298.1948066931273615, -330.5268031993605859 ) ) ;
#15861=CARTESIAN_POINT ( 'NONE',  ( -29.40795054730552494, -281.6345175559641234, -343.4756271270165939 ) ) ;
#15863=CARTESIAN_POINT ( 'NONE',  ( -69.53939256847833406, -275.4747023180252654, -338.2967640226538037 ) ) ;
#15866=CARTESIAN_POINT ( 'NONE',  ( -112.4192724977080502, -294.7835768336193496, -283.6904141885146942 ) ) ;
#15868=CARTESIAN_POINT ( 'NONE',  ( 34.26273633242944072, -275.0946559646685614, -285.0817615718671050 ) ) ;
#15869=CARTESIAN_POINT ( 'NONE',  ( -60.49499394487303050, -293.2666145312089725, -200.3459167165141253 ) ) ;
#15870=CARTESIAN_POINT ( 'NONE',  ( 20.71704865997834588, -295.1198167787104012, -315.0200924110563960 ) ) ;
#15871=CARTESIAN_POINT ( 'NONE',  ( -105.0311366971539826, -285.9149389863769670, -300.2962843925435550 ) ) ;
#15872=CARTESIAN_POINT ( 'NONE',  ( 3.808804004809474453, -294.0193454912460425, -205.9148541086267130 ) ) ;
#15873=CARTESIAN_POINT ( 'NONE',  ( 31.73346565615385728, -294.4415800110484156, -237.3455084458495605 ) ) ;
#15874=CARTESIAN_POINT ( 'NONE',  ( -67.29715047758752178, -295.2895583513290489, -336.9456211854137564 ) ) ;
#15875=CARTESIAN_POINT ( 'NONE',  ( -100.5129852052107395, -292.0079916843238266, -310.7887000235631376 ) ) ;
#15876=CARTESIAN_POINT ( 'NONE',  ( -92.43225546529755832, -283.9808764911872458, -324.1573141040151427 ) ) ;
#15877=CARTESIAN_POINT ( 'NONE',  ( -33.40300596452087944, -296.1809437869289354, -194.8023867302687506 ) ) ;
#15878=CARTESIAN_POINT ( 'NONE',  ( -107.0065457804658564, -283.9653439342915249, -303.1606497583886153 ) ) ;
#15879=CARTESIAN_POINT ( 'NONE',  ( -95.72406915748916845, -279.8894060920168840, -316.8933080821197450 ) ) ;
#15880=CARTESIAN_POINT ( 'NONE',  ( -33.20099175315139206, -284.9002324454621089, -197.0308457171405223 ) ) ;
#15881=CARTESIAN_POINT ( 'NONE',  ( 36.07122548115266625, -285.3541356083511005, -254.9514249164482464 ) ) ;
#15882=CARTESIAN_POINT ( 'NONE',  ( -99.22617866293555267, -277.2795860729529522, -226.6505151729262479 ) ) ;
#15883=CARTESIAN_POINT ( 'NONE',  ( -32.04911714649202992, -124.5213432794980974, -365.6788127701597659 ) ) ;
#15884=CARTESIAN_POINT ( 'NONE',  ( -67.56743679874085728, -285.1522027307956364, -203.8450050131483522 ) ) ;
#15885=CARTESIAN_POINT ( 'NONE',  ( 25.61280253863908030, -283.3369909798606727, -314.0275131697265465 ) ) ;
#15886=CARTESIAN_POINT ( 'NONE',  ( -80.41852276767058072, -288.6787774023308657, -333.9643640420392217 ) ) ;
#15887=CARTESIAN_POINT ( 'NONE',  ( -98.99041047885765465, -279.5515372482508383, -315.1703149527498340 ) ) ;
#15888=CARTESIAN_POINT ( 'NONE',  ( -96.66133552830895326, -279.2145446872268622, -318.6980759225766633 ) ) ;
#15889=CARTESIAN_POINT ( 'NONE',  ( -39.69910605584753682, -279.8550781085256745, -197.3866722092923851 ) ) ;
#15890=CARTESIAN_POINT ( 'NONE',  ( -4.609045273264730902, -276.4653987453200443, -203.2618146295105248 ) ) ;
#15891=CARTESIAN_POINT ( 'NONE',  ( 35.45261220471979868, -293.2339486485220732, -245.1001564367266212 ) ) ;
#15892=CARTESIAN_POINT ( 'NONE',  ( -11.36221711908693699, -284.3912514542772669, -200.1820976934847067 ) ) ;
#15893=CARTESIAN_POINT ( 'NONE',  ( 3.693376998837470726, -294.1941734058470388, -206.0913973756002804 ) ) ;
#15894=CARTESIAN_POINT ( 'NONE',  ( -4.209203439874178443, -293.5250542679443129, -335.7698510459715635 ) ) ;
#15895=CARTESIAN_POINT ( 'NONE',  ( 16.17174615579032704, -293.9327703463718535, -320.0440985052070459 ) ) ;
#15896=CARTESIAN_POINT ( 'NONE',  ( -109.1891016106313685, -291.9741175021994763, -243.3872642888283622 ) ) ;
#15898=CARTESIAN_POINT ( 'NONE',  ( 26.54390395016679349, -281.7184280983207145, -234.8291287410467021 ) ) ;
#15899=CARTESIAN_POINT ( 'NONE',  ( -23.41573227742476604, -297.1429999092800927, -193.6727113408300909 ) ) ;
#15900=CARTESIAN_POINT ( 'NONE',  ( 38.18850224560330986, -288.0227361338855303, -255.9215433258822827 ) ) ;
#15901=CARTESIAN_POINT ( 'NONE',  ( 6.195537895881389368, -280.6081295510135192, -332.4318260222510730 ) ) ;
#15902=CARTESIAN_POINT ( 'NONE',  ( -70.62608484619411797, -289.8123273752514137, -339.7866506870747685 ) ) ;
#15903=CARTESIAN_POINT ( 'NONE',  ( -65.10519041269610341, -286.0125392203438537, -202.7700729462104050 ) ) ;
#15905=CARTESIAN_POINT ( 'NONE',  ( -90.98605276365739769, -229.1079664473872413, -346.1131341628189375 ) ) ;
#15906=CARTESIAN_POINT ( 'NONE',  ( 45.01749665140694390, 11.19730123446569081, -328.3103152587933664 ) ) ;
#15908=CARTESIAN_POINT ( 'NONE',  ( -68.58298753371472856, -278.8278934792664927, -204.2053647272176988 ) ) ;
#15909=CARTESIAN_POINT ( 'NONE',  ( -109.1874494767653516, -277.6647556635431897, -255.7236955823417475 ) ) ;
#15910=CARTESIAN_POINT ( 'NONE',  ( -113.0467096792613972, -272.3968957623358165, -256.1304345755483496 ) ) ;
#15911=CARTESIAN_POINT ( 'NONE',  ( -81.55632558770187757, -219.7645460677553899, -349.7766062465405525 ) ) ;
#15912=CARTESIAN_POINT ( 'NONE',  ( -35.33318618733856908, -278.6516012964420383, -193.9637106765003693 ) ) ;
#15913=CARTESIAN_POINT ( 'NONE',  ( 14.79984501326969237, -296.0895561520632668, -325.6352826736072643 ) ) ;
#15915=CARTESIAN_POINT ( 'NONE',  ( -47.00880822376538504, -292.4183950030986239, -197.9419529595729728 ) ) ;
#15916=CARTESIAN_POINT ( 'NONE',  ( -33.35518257146905796, -298.9037006361731414, -193.5220654726613816 ) ) ;
#15917=CARTESIAN_POINT ( 'NONE',  ( -31.85111590134202686, -287.6663828040902899, -343.6998511869097115 ) ) ;
#15918=CARTESIAN_POINT ( 'NONE',  ( -20.53292325580157041, -298.7496616662710949, -193.4212930106775161 ) ) ;
#15919=CARTESIAN_POINT ( 'NONE',  ( -108.1754613256751867, -296.9523789220810386, -252.6583560709639187 ) ) ;
#15922=CARTESIAN_POINT ( 'NONE',  ( -38.17894846926897401, -281.9618848822379391, -194.8057527372322966 ) ) ;
#15924=CARTESIAN_POINT ( 'NONE',  ( -109.5883790293937778, -279.4674996136322420, -282.8708092280111259 ) ) ;
#15925=CARTESIAN_POINT ( 'NONE',  ( -79.64321512363108013, -279.3750100342851397, -333.5477849375291726 ) ) ;
#15926=CARTESIAN_POINT ( 'NONE',  ( -85.75117965112542606, -271.8478354881674477, -214.7302729333593163 ) ) ;
#15929=CARTESIAN_POINT ( 'NONE',  ( 26.45781019393561806, -281.2337729652594476, -234.8840481041486896 ) ) ;
#15930=CARTESIAN_POINT ( 'NONE',  ( 36.73268832053429378, -276.6119308294917118, -290.8343009444925542 ) ) ;
#15931=CARTESIAN_POINT ( 'NONE',  ( -6.094197931968958315, -278.6416711544894156, -338.5417182950293977 ) ) ;
#15932=CARTESIAN_POINT ( 'NONE',  ( -56.79170282384747281, -275.8727652911543942, -344.3096208910608880 ) ) ;
#15935=CARTESIAN_POINT ( 'NONE',  ( -22.03492582838287106, -284.8368732810368442, -344.1453267289542737 ) ) ;
#15936=CARTESIAN_POINT ( 'NONE',  ( -36.19336221950214849, -291.2640432893157367, -197.1961496731574641 ) ) ;
#15937=CARTESIAN_POINT ( 'NONE',  ( -54.93322377169864268, -285.1802831239406828, -195.5022435442901099 ) ) ;
#15938=CARTESIAN_POINT ( 'NONE',  ( -92.43411711634762185, -282.0941886324004031, -319.8048815337610336 ) ) ;
#15939=CARTESIAN_POINT ( 'NONE',  ( -78.72283324967605722, -282.1966108107049536, -331.2132069982210965 ) ) ;
#15940=CARTESIAN_POINT ( 'NONE',  ( -38.37478025898267475, -281.2439995241444990, -196.9588460392263585 ) ) ;
#15941=CARTESIAN_POINT ( 'NONE',  ( 84.21812863670487559, 83.45443854015287855, -302.1763853752734690 ) ) ;
#15942=CARTESIAN_POINT ( 'NONE',  ( -68.87420532806851270, -281.8597041497235978, -339.7449853301349094 ) ) ;
#15943=CARTESIAN_POINT ( 'NONE',  ( 23.28500189172707380, -296.1541468748567354, -314.5348119044927557 ) ) ;
#15944=CARTESIAN_POINT ( 'NONE',  ( -104.3615276920238699, -278.8100721612821076, -299.6809964782769384 ) ) ;
#15945=CARTESIAN_POINT ( 'NONE',  ( -46.31257577213033017, -287.9387348551020409, -195.7316880277365101 ) ) ;
#15947=CARTESIAN_POINT ( 'NONE',  ( -100.4941334670849642, -293.0291063376437819, -228.7812293942942006 ) ) ;
#15948=CARTESIAN_POINT ( 'NONE',  ( 33.99278675747681433, -273.8510802729205125, -293.5212481501260413 ) ) ;
#15949=CARTESIAN_POINT ( 'NONE',  ( -12.28606465868557329, -287.9316237590953165, -343.0555225710816103 ) ) ;
#15950=CARTESIAN_POINT ( 'NONE',  ( -30.71506785053314914, -290.5371847694526650, -196.8592257636908300 ) ) ;
#15951=CARTESIAN_POINT ( 'NONE',  ( -109.2507453764554413, -277.0381129366954269, -285.5378334026153766 ) ) ;
#15952=CARTESIAN_POINT ( 'NONE',  ( -110.2544665096139624, -294.8735690269878091, -256.3438328149949825 ) ) ;
#15953=CARTESIAN_POINT ( 'NONE',  ( -110.8299773619172015, -291.8562414405818686, -271.2076318766708596 ) ) ;
#15956=CARTESIAN_POINT ( 'NONE',  ( 39.01782031851747945, -292.0316349883576663, -270.3297410190102710 ) ) ;
#15957=CARTESIAN_POINT ( 'NONE',  ( 15.58923712835949082, -288.4167404178641618, -218.9339238530691318 ) ) ;
#15958=CARTESIAN_POINT ( 'NONE',  ( -94.70820682386745659, -288.1095375210364296, -320.1914092210054719 ) ) ;
#15959=CARTESIAN_POINT ( 'NONE',  ( -10.49233490484472853, -290.1202742494306790, -338.9321004164506803 ) ) ;
#15961=CARTESIAN_POINT ( 'NONE',  ( 28.37728414301563973, -288.7895063551759449, -302.5110298454625308 ) ) ;
#15962=CARTESIAN_POINT ( 'NONE',  ( -34.88251444973987958, -297.0012882059284607, -345.6761842802283127 ) ) ;
#15964=CARTESIAN_POINT ( 'NONE',  ( -41.72243194040052572, -290.3112279792222239, -346.8518367590256730 ) ) ;
#15965=CARTESIAN_POINT ( 'NONE',  ( -111.1022407369145526, -276.7701167893360434, -254.8785703103167464 ) ) ;
#15966=CARTESIAN_POINT ( 'NONE',  ( -112.3820702055426466, -279.1001805600450325, -253.1946637674726901 ) ) ;
#15967=CARTESIAN_POINT ( 'NONE',  ( -48.11162366469079643, -279.5855622687032564, -194.0855526428520363 ) ) ;
#15968=CARTESIAN_POINT ( 'NONE',  ( -107.4250137091842703, -282.8990944422551479, -243.6528832169257157 ) ) ;
#15970=CARTESIAN_POINT ( 'NONE',  ( -82.01258227717343630, -277.5758828579101873, -211.0059641890439366 ) ) ;
#15972=CARTESIAN_POINT ( 'NONE',  ( -107.4429284448295761, -282.2038508074141419, -297.1671448048194293 ) ) ;
#15973=CARTESIAN_POINT ( 'NONE',  ( 26.24832811123609133, -24.45034257384636334, -341.6199305999596163 ) ) ;
#15974=CARTESIAN_POINT ( 'NONE',  ( -105.5470917296300115, -277.4775168405614068, -236.0275290323528168 ) ) ;
#15975=AXIS2_PLACEMENT_3D ( 'NONE', #91706, #26858, #12666 ) ;
#15976=CARTESIAN_POINT ( 'NONE',  ( -37.84651135024520840, -299.5658396127653305, -196.6695111315174813 ) ) ;
#15977=CARTESIAN_POINT ( 'NONE',  ( -105.5156940864888071, -283.0166399422415111, -305.6025031000589820 ) ) ;
#15978=CARTESIAN_POINT ( 'NONE',  ( -78.95529992700123501, -274.2782271399448177, -210.1255761164408113 ) ) ;
#15979=CARTESIAN_POINT ( 'NONE',  ( -57.98005124871750127, -275.2160329142224100, -196.7352989101937339 ) ) ;
#15980=CARTESIAN_POINT ( 'NONE',  ( 33.85532700170085718, -275.0043060808779956, -254.0857411769362670 ) ) ;
#15981=CARTESIAN_POINT ( 'NONE',  ( -70.58835413796140301, -297.4907178387658178, -337.5895394291843559 ) ) ;
#15982=CARTESIAN_POINT ( 'NONE',  ( -31.82465905316621857, -289.1511588016697942, -347.2157719042038480 ) ) ;
#15983=CARTESIAN_POINT ( 'NONE',  ( -20.06133236464767577, -278.3522344582344203, -196.7498858325006097 ) ) ;
#15984=CARTESIAN_POINT ( 'NONE',  ( -113.6658509090508176, -290.5176634014234764, -259.7912570798114302 ) ) ;
#15985=CARTESIAN_POINT ( 'NONE',  ( -23.75323706710615923, -287.9331266285080346, -342.3765984985037107 ) ) ;
#15986=CARTESIAN_POINT ( 'NONE',  ( 24.84913480755347237, -290.9838813688306232, -228.3495466137204630 ) ) ;
#15989=CARTESIAN_POINT ( 'NONE',  ( -110.3681053163185339, -290.0130823218111686, -273.9056959723057503 ) ) ;
#15991=CARTESIAN_POINT ( 'NONE',  ( 26.15597618984440942, -287.9226188571277589, -227.1998933662609943 ) ) ;
#15992=CARTESIAN_POINT ( 'NONE',  ( -53.35057174420112602, -288.3376638359845288, -200.3683826091709648 ) ) ;
#15993=CARTESIAN_POINT ( 'NONE',  ( -71.97862873181199461, -294.5576543056366177, -338.8673468289770767 ) ) ;
#15994=CARTESIAN_POINT ( 'NONE',  ( -27.41935687340967931, -284.2439015776776046, -346.2748353269673771 ) ) ;
#15995=CARTESIAN_POINT ( 'NONE',  ( -81.47688983342892755, -285.2656708238984606, -212.2140197389120715 ) ) ;
#15996=CARTESIAN_POINT ( 'NONE',  ( 14.08831880860145880, -277.6270861099894773, -322.9315021422164023 ) ) ;
#15997=CARTESIAN_POINT ( 'NONE',  ( 37.17842697681656716, -291.5060297671319631, -265.2277950931076589 ) ) ;
#15998=CARTESIAN_POINT ( 'NONE',  ( -13.92430640745994808, -273.1578094841852931, -200.7999493921857095 ) ) ;
#16001=CARTESIAN_POINT ( 'NONE',  ( 8.890071546132155333, -294.1039135029694762, -331.9108343044175058 ) ) ;
#16002=CARTESIAN_POINT ( 'NONE',  ( -1.514382050981514460, -288.4507612945305368, -205.0521037722574533 ) ) ;
#16003=CARTESIAN_POINT ( 'NONE',  ( -111.9767195722728133, -297.8533098234541967, -252.7229099152794447 ) ) ;
#16004=CARTESIAN_POINT ( 'NONE',  ( 35.65388830598798364, -288.1404780496431499, -265.5717704489886160 ) ) ;
#16005=CARTESIAN_POINT ( 'NONE',  ( -95.97724669800747677, -276.9411765550994460, -319.9262680029857506 ) ) ;
#16006=CARTESIAN_POINT ( 'NONE',  ( 38.22352988415124031, -294.0250459441383555, -256.1059855716057427 ) ) ;
#16007=CARTESIAN_POINT ( 'NONE',  ( 33.70432100556923416, -285.3535576477246423, -244.0406248269138132 ) ) ;
#16008=CARTESIAN_POINT ( 'NONE',  ( -5.802482194022864803, -294.9819628773301474, -340.5823542556489087 ) ) ;
#16009=CARTESIAN_POINT ( 'NONE',  ( -30.80930709945117840, -292.4702824665305911, -197.6327512465219911 ) ) ;
#16012=CARTESIAN_POINT ( 'NONE',  ( 121.9599628496891199, 147.3134478266455858, -260.3665198286096256 ) ) ;
#16013=CARTESIAN_POINT ( 'NONE',  ( 37.15234745078601719, -289.2816694478893851, -286.9539744732303461 ) ) ;
#16014=CARTESIAN_POINT ( 'NONE',  ( 40.64545035920995986, -291.2666405000203440, -288.1938231032136741 ) ) ;
#16016=CARTESIAN_POINT ( 'NONE',  ( -7.138634476440246068, -281.5666852245482232, -337.1730985148406035 ) ) ;
#16018=CARTESIAN_POINT ( 'NONE',  ( -99.40830359821914897, -278.8240376995777297, -224.8033809663859017 ) ) ;
#16019=CARTESIAN_POINT ( 'NONE',  ( -2.312924976743116812, -282.5169013330373105, -204.2178230401108294 ) ) ;
#16020=CARTESIAN_POINT ( 'NONE',  ( 140.7620216225690513, 178.5875772026313655, -240.1871175959595917 ) ) ;
#16021=CARTESIAN_POINT ( 'NONE',  ( -110.9289524669257503, -282.8670230415570472, -290.9407823859006612 ) ) ;
#16022=CARTESIAN_POINT ( 'NONE',  ( -14.02889745157004597, -284.3760360332855726, -199.3959674231889210 ) ) ;
#16023=CARTESIAN_POINT ( 'NONE',  ( -1.900611152839966067, -276.3769347467678017, -203.3966894039688214 ) ) ;
#16024=CARTESIAN_POINT ( 'NONE',  ( -37.15574612518469166, -298.5468983951584505, -197.2967118480558781 ) ) ;
#16025=CARTESIAN_POINT ( 'NONE',  ( -7.805381360236214761, -293.3416322997192651, -337.6715115575364052 ) ) ;
#16026=CARTESIAN_POINT ( 'NONE',  ( -114.1297772558595369, -279.1520765492772398, -274.4725650905581915 ) ) ;
#16027=CARTESIAN_POINT ( 'NONE',  ( 13.73132837925489191, -276.3121239811382566, -322.5903691034905023 ) ) ;
#16028=CARTESIAN_POINT ( 'NONE',  ( -97.57884793293831649, -274.2691969759052313, -222.8955669411934082 ) ) ;
#16029=CARTESIAN_POINT ( 'NONE',  ( -34.31710452439213554, -275.9352915484344066, -346.9923409395666454 ) ) ;
#16030=CARTESIAN_POINT ( 'NONE',  ( 44.71985729433082923, 12.68782823267609317, -331.8881429784909756 ) ) ;
#16031=CARTESIAN_POINT ( 'NONE',  ( 37.45749664270536528, -273.4730664455656779, -264.2145073729544151 ) ) ;
#16032=CARTESIAN_POINT ( 'NONE',  ( -79.13936011121289482, -297.0295013246803819, -334.3264360214186581 ) ) ;
#16033=CARTESIAN_POINT ( 'NONE',  ( 35.77081079830085031, -277.8376638359845288, -253.6410175316879361 ) ) ;
#16034=CARTESIAN_POINT ( 'NONE',  ( -75.88346903603265048, -208.4961600436150491, -353.2410745688453062 ) ) ;
#16035=CARTESIAN_POINT ( 'NONE',  ( -92.78392803130417121, -284.9511082673145665, -318.3425501721818023 ) ) ;
#16036=CARTESIAN_POINT ( 'NONE',  ( -96.37083773251768548, -285.6617165488259502, -318.2306435912695406 ) ) ;
#16037=CARTESIAN_POINT ( 'NONE',  ( -79.49530807252376974, -277.8719472713040091, -209.7846064390230936 ) ) ;
#16038=CARTESIAN_POINT ( 'NONE',  ( -94.21645785844144427, -287.0787547989395989, -222.6523408437553542 ) ) ;
#16039=CARTESIAN_POINT ( 'NONE',  ( -70.03057599244034748, -278.0933810515128926, -204.3006055294051464 ) ) ;
#16040=CARTESIAN_POINT ( 'NONE',  ( 29.44149659727181856, -277.0376205212172067, -300.5973662254262422 ) ) ;
#16042=CARTESIAN_POINT ( 'NONE',  ( -63.33447121381287559, -274.1965124705897097, -202.0661048834799658 ) ) ;
#16044=CARTESIAN_POINT ( 'NONE',  ( 27.70918862855555886, -281.8172271736654011, -229.3647172867792960 ) ) ;
#16045=CARTESIAN_POINT ( 'NONE',  ( 39.21753779596305378, -282.1464396975984528, -278.5057770675436473 ) ) ;
#16046=ORIENTED_EDGE ( 'NONE', *, *, #85141, .T. ) ;
#16049=CARTESIAN_POINT ( 'NONE',  ( 37.74787919503628331, -289.2842867356879424, -260.2685188536830765 ) ) ;
#16050=CARTESIAN_POINT ( 'NONE',  ( -110.3728692653498769, -295.8067645240708430, -265.9964804282588489 ) ) ;
#16051=CARTESIAN_POINT ( 'NONE',  ( -44.87878834859591848, -291.3078362498685010, -193.7804598259594115 ) ) ;
#16052=CARTESIAN_POINT ( 'NONE',  ( 30.05134854030556824, -286.4309944584211962, -300.3018195713866021 ) ) ;
#16053=CARTESIAN_POINT ( 'NONE',  ( -73.85295584869059837, -288.1218602330084195, -334.2685510387424870 ) ) ;
#16054=CARTESIAN_POINT ( 'NONE',  ( 2.650589609416499570, -287.8068680873333278, -208.8164409923248002 ) ) ;
#16055=CARTESIAN_POINT ( 'NONE',  ( -98.84052424263423120, -275.9694145365216968, -313.2900742052197529 ) ) ;
#16056=CARTESIAN_POINT ( 'NONE',  ( -5.974618698033269837, -287.0465638603076854, -339.8056758700995488 ) ) ;
#16057=CARTESIAN_POINT ( 'NONE',  ( 35.42991462233113253, -289.3192266963542352, -252.2146930160136833 ) ) ;
#16058=CARTESIAN_POINT ( 'NONE',  ( -36.14226692367611804, -287.0370230906651159, -345.5310172501127681 ) ) ;
#16059=CARTESIAN_POINT ( 'NONE',  ( -37.52912586339792256, -283.9958444141489622, -343.6086424470119027 ) ) ;
#16060=CARTESIAN_POINT ( 'NONE',  ( -100.7409079118262980, -292.0089555227912115, -310.8371557114539883 ) ) ;
#16061=CARTESIAN_POINT ( 'NONE',  ( 82.17387051439972367, -297.5899665652531212, -194.8765235847432109 ) ) ;
#16063=CARTESIAN_POINT ( 'NONE',  ( -36.23581135676069920, -299.9860413745942083, -194.8007515470732187 ) ) ;
#16064=CARTESIAN_POINT ( 'NONE',  ( 15.38283133894301891, -280.0178999546803880, -219.5666926775269303 ) ) ;
#16065=CARTESIAN_POINT ( 'NONE',  ( 35.25312124887982890, -279.7946907519416300, -289.2534509245011805 ) ) ;
#16066=CARTESIAN_POINT ( 'NONE',  ( 37.60607962888355615, -292.5363440170551712, -253.3613360465822382 ) ) ;
#16067=CARTESIAN_POINT ( 'NONE',  ( -40.53238431738569147, -296.4112665006975931, -196.6174343441556118 ) ) ;
#16068=CARTESIAN_POINT ( 'NONE',  ( -4.451425840511100240, -274.6952289539471508, -337.1550983218368742 ) ) ;
#16069=CARTESIAN_POINT ( 'NONE',  ( -96.79757616207875515, -297.2665270595649076, -313.5826181306987905 ) ) ;
#16071=CARTESIAN_POINT ( 'NONE',  ( -64.67224439009181935, -272.2769405454720300, -198.9912602122829810 ) ) ;
#16072=CARTESIAN_POINT ( 'NONE',  ( -95.74712210801881440, -294.1293270918399685, -318.9898003738420016 ) ) ;
#16073=CARTESIAN_POINT ( 'NONE',  ( 27.68719393287989305, -295.4442033218020356, -304.9173770732336379 ) ) ;
#16076=CARTESIAN_POINT ( 'NONE',  ( -5.461923765841955714, -295.4245150839213352, -336.2254089208943242 ) ) ;
#16077=FACE_OUTER_BOUND ( 'NONE', #57601, .T. ) ;
#16078=CARTESIAN_POINT ( 'NONE',  ( -102.6030942302557065, -283.0739400894740356, -232.5830511604771971 ) ) ;
#16079=CARTESIAN_POINT ( 'NONE',  ( -107.9695772386578199, -296.3078622881507727, -288.8686819391106724 ) ) ;
#16080=CARTESIAN_POINT ( 'NONE',  ( -110.2246821559504895, -284.2391628523432701, -295.2020304200150349 ) ) ;
#16081=CARTESIAN_POINT ( 'NONE',  ( -60.76167112943635829, -285.2737026592313327, -342.2545956808456822 ) ) ;
#16082=CARTESIAN_POINT ( 'NONE',  ( -95.79772248370970544, -284.8955784066761225, -220.1948713567610696 ) ) ;
#16083=CARTESIAN_POINT ( 'NONE',  ( -58.14066155079859755, -289.7827586593165847, -198.4220689122026897 ) ) ;
#16084=CARTESIAN_POINT ( 'NONE',  ( 21.27581636871891391, -273.6952119285918457, -317.1477375740089997 ) ) ;
#16086=CARTESIAN_POINT ( 'NONE',  ( -25.04291726254466255, -284.8969545776492396, -197.8527026799237660 ) ) ;
#16087=CARTESIAN_POINT ( 'NONE',  ( -97.05808429791169090, -288.8246426337437356, -318.5009133096664868 ) ) ;
#16088=DIRECTION ( 'NONE',  ( 1.000000000000000000, 0.000000000000000000, 0.000000000000000000 ) ) ;
#16089=CARTESIAN_POINT ( 'NONE',  ( -109.5662386839992166, -298.3509779018197037, -255.1326617795067762 ) ) ;
#16090=CARTESIAN_POINT ( 'NONE',  ( -113.1791059691529284, -279.8544022416588746, -280.1223710940091678 ) ) ;
#16091=CARTESIAN_POINT ( 'NONE',  ( -61.09747669634701595, -293.3790022065677476, -341.9283988016326816 ) ) ;
#16092=CARTESIAN_POINT ( 'NONE',  ( 17.08140358048866148, -280.5225550356768167, -221.6762818470592151 ) ) ;
#16093=CARTESIAN_POINT ( 'NONE',  ( -11.05521348601741671, -294.8856093736546313, -342.7918589543522785 ) ) ;
#16094=CARTESIAN_POINT ( 'NONE',  ( -80.10275740121561228, -283.5585783044428467, -208.0018590886799643 ) ) ;
#16096=CARTESIAN_POINT ( 'NONE',  ( -72.84204861055374636, -281.5820908615443159, -204.2804810407856166 ) ) ;
#16097=CARTESIAN_POINT ( 'NONE',  ( -59.53141437658843671, -295.7647791016218548, -198.6647581677904952 ) ) ;
#16100=CARTESIAN_POINT ( 'NONE',  ( -4.865155017680591776, -282.4618619047147945, -203.1515887103534510 ) ) ;
#16101=CARTESIAN_POINT ( 'NONE',  ( -63.59695877118431895, -294.9113420021631100, -338.5957313310985910 ) ) ;
#16103=CARTESIAN_POINT ( 'NONE',  ( -114.2704648735229114, -276.0523547857348490, -270.3284710469133074 ) ) ;
#16104=CARTESIAN_POINT ( 'NONE',  ( -81.14991594156447263, -272.6709884484788518, -207.1697987114992259 ) ) ;
#16105=CARTESIAN_POINT ( 'NONE',  ( -69.01568047157188346, -291.4570071418833663, -204.5768126635960868 ) ) ;
#16106=CARTESIAN_POINT ( 'NONE',  ( -66.36038006800242783, -281.1853093273176682, -202.6079648835188038 ) ) ;
#16107=CARTESIAN_POINT ( 'NONE',  ( -83.70885577685095313, -275.0035149987531327, -212.9457255338397772 ) ) ;
#16108=CARTESIAN_POINT ( 'NONE',  ( -38.69766541833456586, -284.6690149806497061, -346.5490551911209423 ) ) ;
#16110=CARTESIAN_POINT ( 'NONE',  ( -94.23866423185275210, -277.9998722057171676, -223.9944706818797329 ) ) ;
#16111=CARTESIAN_POINT ( 'NONE',  ( -41.95483215792304321, -279.1104285126171476, -345.2320561957508289 ) ) ;
#16113=CARTESIAN_POINT ( 'NONE',  ( -63.55509974514872340, -273.5530578305539393, -197.9604433654228046 ) ) ;
#16114=CARTESIAN_POINT ( 'NONE',  ( -44.46181446769116974, -293.8816772640726640, -196.2105912024025258 ) ) ;
#16117=CARTESIAN_POINT ( 'NONE',  ( -34.91826982551637570, -293.1616009775517000, -346.0871535881247496 ) ) ;
#16118=CARTESIAN_POINT ( 'NONE',  ( -52.63537675050562825, -297.5176346686349689, -198.9076008994401548 ) ) ;
#16120=CARTESIAN_POINT ( 'NONE',  ( -19.56723662603547709, -293.7967052494137192, -196.0991370707760382 ) ) ;
#16121=CARTESIAN_POINT ( 'NONE',  ( -106.6662871844225293, -275.4805209788417528, -237.0123917617630980 ) ) ;
#16122=CARTESIAN_POINT ( 'NONE',  ( 21.77363748050969150, -288.9218133094374252, -224.4764223860316008 ) ) ;
#16123=CARTESIAN_POINT ( 'NONE',  ( 25.51069872189556165, -274.1016340840220664, -311.0719376254648978 ) ) ;
#16124=CARTESIAN_POINT ( 'NONE',  ( 36.26187065873975257, -277.3272472470691241, -259.1477087954085050 ) ) ;
#16125=CARTESIAN_POINT ( 'NONE',  ( -4.936319404313901593, -292.7019694950465123, -337.3916552285003263 ) ) ;
#16126=CARTESIAN_POINT ( 'NONE',  ( -76.86865594529287193, -281.3896297829937794, -205.6635001278857544 ) ) ;
#16128=CARTESIAN_POINT ( 'NONE',  ( -10.97209389845760619, -282.3655270742172547, -338.5082610651087975 ) ) ;
#16129=CARTESIAN_POINT ( 'NONE',  ( -107.2885073356802792, -279.2270999094243962, -301.9376500331092643 ) ) ;
#16130=CARTESIAN_POINT ( 'NONE',  ( 1.877597072067028749, -281.3345076314728317, -336.1627550862185672 ) ) ;
#16131=CARTESIAN_POINT ( 'NONE',  ( -54.06826681389222955, -278.2029686009424836, -345.3358283903361325 ) ) ;
#16132=CARTESIAN_POINT ( 'NONE',  ( 38.05380001206331997, -277.2248352481663005, -282.4502466002586516 ) ) ;
#16133=CARTESIAN_POINT ( 'NONE',  ( 17.36665895637874613, -283.4090924074130839, -226.6919474004047572 ) ) ;
#16135=CARTESIAN_POINT ( 'NONE',  ( -104.3298507207468475, -298.9992136834750909, -236.5172525613756704 ) ) ;
#16136=CARTESIAN_POINT ( 'NONE',  ( -109.5837590857027806, -291.7993450544401526, -257.6085902228123814 ) ) ;
#16137=CARTESIAN_POINT ( 'NONE',  ( -111.2467396229617691, -276.7121135475974256, -259.5203760085709064 ) ) ;
#16138=CARTESIAN_POINT ( 'NONE',  ( -105.5933421259349956, -291.8762641739260175, -303.8825561424387161 ) ) ;
#16139=CARTESIAN_POINT ( 'NONE',  ( -67.83615987349411114, -290.9896026955631214, -203.9095704579743540 ) ) ;
#16140=CARTESIAN_POINT ( 'NONE',  ( 38.23091782796835503, -286.8791606111798274, -255.9282970985375414 ) ) ;
#16142=CARTESIAN_POINT ( 'NONE',  ( -111.1194504936760552, -282.9090520012756542, -273.6537263002545615 ) ) ;
#16143=CARTESIAN_POINT ( 'NONE',  ( -111.2042228462525912, -292.5089467253582711, -262.9319042489740355 ) ) ;
#16144=CARTESIAN_POINT ( 'NONE',  ( -65.33886147741188211, -284.1594353396785664, -202.1388762867762807 ) ) ;
#16145=CARTESIAN_POINT ( 'NONE',  ( 34.97368775861869494, -283.0399653335376229, -283.5362312299162681 ) ) ;
#16146=CARTESIAN_POINT ( 'NONE',  ( -73.05374079550901456, -290.4549140917231398, -338.3277993792888196 ) ) ;
#16147=CARTESIAN_POINT ( 'NONE',  ( -97.69613262048412139, -278.4721298600538262, -311.5355143986197390 ) ) ;
#16148=CARTESIAN_POINT ( 'NONE',  ( -58.81261158464429428, -290.5753408759996432, -196.8287531433772983 ) ) ;
#16149=CARTESIAN_POINT ( 'NONE',  ( 39.47839147570288532, -288.3338913960093919, -268.6781604700288426 ) ) ;
#16150=CARTESIAN_POINT ( 'NONE',  ( 35.01673811254666191, -288.3767458938384607, -296.6654093139031829 ) ) ;
#16151=CARTESIAN_POINT ( 'NONE',  ( -10.75194963637617995, -286.5754825251138413, -202.3624088034963791 ) ) ;
#16155=CARTESIAN_POINT ( 'NONE',  ( -40.60334466124434982, -293.8719852272722619, -194.6535824823055236 ) ) ;
#16156=CARTESIAN_POINT ( 'NONE',  ( -110.3343596821110850, -294.9466120360130503, -293.3259483935088383 ) ) ;
#16157=CARTESIAN_POINT ( 'NONE',  ( -70.57023658465119809, -276.5603056892726954, -335.6242225191335251 ) ) ;
#16158=CARTESIAN_POINT ( 'NONE',  ( -36.88926682509398347, -297.4062679019811526, -193.4630985363918114 ) ) ;
#16159=CARTESIAN_POINT ( 'NONE',  ( 16.65409918822919266, -292.7461211028290791, -320.5125028983997026 ) ) ;
#16160=CARTESIAN_POINT ( 'NONE',  ( -110.2705752990698471, -294.9562527459866033, -257.7376010002607245 ) ) ;
#16161=CARTESIAN_POINT ( 'NONE',  ( -75.19748937292605717, -292.7409352337436985, -207.4203806474900489 ) ) ;
#16162=CARTESIAN_POINT ( 'NONE',  ( 35.84231423949732687, -294.5651007754024704, -265.2812828875474906 ) ) ;
#16164=CARTESIAN_POINT ( 'NONE',  ( 5.546545866062435159, -292.4731416880759411, -332.1547990540379942 ) ) ;
#16166=CARTESIAN_POINT ( 'NONE',  ( -92.58133364584938363, -290.8093285287337721, -318.5200577232094474 ) ) ;
#16167=CARTESIAN_POINT ( 'NONE',  ( -45.08875949535130445, -295.4861018686797252, -343.0206345511993504 ) ) ;
#16168=CARTESIAN_POINT ( 'NONE',  ( -3.441966035370155996, -278.5868235652208682, -337.6749259665084537 ) ) ;
#16169=CARTESIAN_POINT ( 'NONE',  ( -59.14547265703046719, -278.4605304936694665, -197.0269937622997816 ) ) ;
#16170=CARTESIAN_POINT ( 'NONE',  ( -104.1368711729147947, -272.3974756500696799, -232.1528593825767643 ) ) ;
#16171=CARTESIAN_POINT ( 'NONE',  ( 35.75279077991758925, -279.4488606623720557, -256.2045091629522062 ) ) ;
#16172=CARTESIAN_POINT ( 'NONE',  ( -112.0138065052718304, -276.7593384483882915, -285.6084693395042109 ) ) ;
#16174=CARTESIAN_POINT ( 'NONE',  ( -104.9136139498326656, -271.5169231970756414, -241.0873924013882004 ) ) ;
#16175=DIRECTION ( 'NONE',  ( -1.000000000000000000, -0.000000000000000000, -0.000000000000000000 ) ) ;
#16176=CARTESIAN_POINT ( 'NONE',  ( -24.58679142903325499, -274.8705162094104821, -198.3288709757293873 ) ) ;
#16178=CARTESIAN_POINT ( 'NONE',  ( -103.7193022270699316, -288.1010246806885675, -306.0321249717113119 ) ) ;
#16179=CARTESIAN_POINT ( 'NONE',  ( -93.59279552133443758, -289.8344171345688096, -323.0194624958240865 ) ) ;
#16180=CARTESIAN_POINT ( 'NONE',  ( 29.60560757263339937, -277.1013848020385808, -236.1838387586753925 ) ) ;
#16181=CARTESIAN_POINT ( 'NONE',  ( -72.50447677735419916, -295.5854839531740481, -204.2889578663002226 ) ) ;
#16182=CARTESIAN_POINT ( 'NONE',  ( -97.05338876062029385, -283.0991579572161072, -318.7416268297466786 ) ) ;
#16184=CARTESIAN_POINT ( 'NONE',  ( -39.31963172620219638, -281.0767920152613897, -345.3475872961309960 ) ) ;
#16186=CARTESIAN_POINT ( 'NONE',  ( -44.32277655854829135, -290.7569513922284159, -197.2457026574006704 ) ) ;
#16187=CARTESIAN_POINT ( 'NONE',  ( -16.80785697581064753, -284.4596247870989032, -198.9685542838419110 ) ) ;
#16189=PLANE ( 'NONE',  #56384 ) ;
#16190=CARTESIAN_POINT ( 'NONE',  ( 37.62112559894191577, -291.5216695801286733, -267.9998884703254589 ) ) ;
#16191=CARTESIAN_POINT ( 'NONE',  ( -72.01218930523641859, -279.1186947887292149, -335.5244118700737204 ) ) ;
#16192=CARTESIAN_POINT ( 'NONE',  ( 17.55250178850824838, -283.4942067149600575, -323.8657153245350173 ) ) ;
#16193=CARTESIAN_POINT ( 'NONE',  ( -66.94844769653154515, -271.7469969881652219, -200.8431009058678001 ) ) ;
#16194=CARTESIAN_POINT ( 'NONE',  ( -97.35594067751075897, -285.1314461345691598, -228.7783325186550769 ) ) ;
#16195=CARTESIAN_POINT ( 'NONE',  ( 31.82173572921842464, -277.3114026359232298, -295.6448123121249409 ) ) ;
#16196=CARTESIAN_POINT ( 'NONE',  ( 3.232133999101723276, -277.2942152897651908, -331.2410466198245445 ) ) ;
#16197=EDGE_CURVE ( 'NONE', #62648, #6475, #75899, .T. ) ;
#16199=CARTESIAN_POINT ( 'NONE',  ( -111.9125248323765192, -286.4494415208300779, -278.3731558253541039 ) ) ;
#16200=B_SPLINE_CURVE_WITH_KNOTS ( 'NONE', 3,
 ( #90920, #24697, #61172, #61627, #4783, #70141, #32738, #4319, #76296, #54975, #41204, #55457, #90460, #33663, #76759, #10471, #47383, #84308, #40736, #46454, #82455, #82907, #19460, #17603, #75815, #39337, #83851, #26086, #68255, #11421 ),
 .UNSPECIFIED., .F., .F.,
 ( 4, 2, 2, 2, 2, 2, 2, 2, 2, 2, 2, 2, 2, 2, 4 ),
 ( 0.006252914598272697050, 0.006643633568813113281, 0.007034352539353530380, 0.007815790480434363710, 0.008206509450974808564, 0.008597228421515255153, 0.008987947392055700008, 0.009378666362596146597, 0.009769385333136593186, 0.01016010430367703804, 0.01055082327421748463, 0.01094154224475792948, 0.01133226121529837607, 0.01172298018583882093, 0.01250441812691963604 ),
 .UNSPECIFIED. ) ;
#16203=CARTESIAN_POINT ( 'NONE',  ( -98.27576076257273030, -295.7571164019763614, -317.4359547759470388 ) ) ;
#16204=CARTESIAN_POINT ( 'NONE',  ( -37.30481570147205161, -288.0324695876779515, -195.7036035952458235 ) ) ;
#16206=CARTESIAN_POINT ( 'NONE',  ( -72.02372285203398405, -289.1237833571631768, -198.2697987213421698 ) ) ;
#16207=CARTESIAN_POINT ( 'NONE',  ( -114.0758385261368204, -277.4570555674865773, -271.5896671702783465 ) ) ;
#16208=CARTESIAN_POINT ( 'NONE',  ( -83.76268854326333724, -289.8271663497507689, -209.8667194249643728 ) ) ;
#16209=CARTESIAN_POINT ( 'NONE',  ( -44.10711869349033520, -287.4851838300175473, -196.9789889320526299 ) ) ;
#16210=CARTESIAN_POINT ( 'NONE',  ( -96.43415456614472703, -280.9299376153308003, -225.7748866482500603 ) ) ;
#16211=CARTESIAN_POINT ( 'NONE',  ( 32.33507018767577534, -289.3811310049298982, -301.7259704401269573 ) ) ;
#16212=CARTESIAN_POINT ( 'NONE',  ( 36.01621212100327796, -283.3511463465368365, -254.6917799651908751 ) ) ;
#16213=CARTESIAN_POINT ( 'NONE',  ( 24.36893000848480284, -276.3314503300293836, -316.4132420668246368 ) ) ;
#16214=CARTESIAN_POINT ( 'NONE',  ( -100.8225511167938748, -271.0855457991739286, -230.7352428114152190 ) ) ;
#16215=CARTESIAN_POINT ( 'NONE',  ( -99.42660992820020738, -278.9906119139737939, -224.7925820697931556 ) ) ;
#16216=CARTESIAN_POINT ( 'NONE',  ( -40.60509971707764265, -299.9309800837078228, -195.9798848392087791 ) ) ;
#16218=CARTESIAN_POINT ( 'NONE',  ( 21.27581636871892101, -277.4090924074130839, -223.5744983911110353 ) ) ;
#16219=CARTESIAN_POINT ( 'NONE',  ( 4.326475101195915940, -272.8451434100428514, -206.7554865447235102 ) ) ;
#16221=CARTESIAN_POINT ( 'NONE',  ( -66.08814367457807748, -279.1731653676085330, -203.1787966177181772 ) ) ;
#16222=CARTESIAN_POINT ( 'NONE',  ( 11.52055205328863252, -275.9173801307104554, -211.2965318148598044 ) ) ;
#16223=CARTESIAN_POINT ( 'NONE',  ( 30.86258623263275069, -281.0663989921815187, -305.5888845073152424 ) ) ;
#16224=CARTESIAN_POINT ( 'NONE',  ( -70.40525860662425828, -291.2542283555349059, -336.5928013246248156 ) ) ;
#16225=CARTESIAN_POINT ( 'NONE',  ( -91.16036202305879499, -298.8240437947548571, -216.2662070974320727 ) ) ;
#16226=CARTESIAN_POINT ( 'NONE',  ( -75.59499989865737746, -298.7590619768773763, -203.9323675152541568 ) ) ;
#16227=CARTESIAN_POINT ( 'NONE',  ( -67.32135804686434710, -293.6582444485196106, -201.7954666681785625 ) ) ;
#16228=CARTESIAN_POINT ( 'NONE',  ( 36.37741274987858020, -279.3864321965698423, -257.4956283005761293 ) ) ;
#16229=CARTESIAN_POINT ( 'NONE',  ( 35.74345521235762391, -283.2885479010608378, -256.1563880442284926 ) ) ;
#16230=CARTESIAN_POINT ( 'NONE',  ( -90.39384897476784886, -271.3166666430514056, -217.8509636826366886 ) ) ;
#16231=CARTESIAN_POINT ( 'NONE',  ( -85.02828893770877983, -287.0065637658222499, -210.9268714483122551 ) ) ;
#16232=CARTESIAN_POINT ( 'NONE',  ( -8.107814036573927297, -287.5804713050972055, -337.6433954937228918 ) ) ;
#16233=CARTESIAN_POINT ( 'NONE',  ( 186.7139198192865592, 262.6718262295162276, -153.2124302575201682 ) ) ;
#16234=VERTEX_POINT ( 'NONE', #2680 ) ;
#16235=CARTESIAN_POINT ( 'NONE',  ( 2.854613614107779807, -287.0990706900261102, -335.4067355553528387 ) ) ;
#16236=CARTESIAN_POINT ( 'NONE',  ( -68.77092333638108812, -289.1438262966360639, -336.2723568982559641 ) ) ;
#16238=CARTESIAN_POINT ( 'NONE',  ( -106.4067259682112194, -286.0612920057370161, -237.0217311469999117 ) ) ;
#16239=CARTESIAN_POINT ( 'NONE',  ( 27.87826845832727329, -275.4398567214372520, -237.5214592713778927 ) ) ;
#16240=CARTESIAN_POINT ( 'NONE',  ( 25.45361613320665128, -293.0572667345268769, -314.4094868430897236 ) ) ;
#16241=CARTESIAN_POINT ( 'NONE',  ( 39.51818539664289176, -282.2339068755487119, -272.7840879383237507 ) ) ;
#16242=CARTESIAN_POINT ( 'NONE',  ( 39.01653097125057457, -283.0666411534982103, -269.9148259015853455 ) ) ;
#16243=CARTESIAN_POINT ( 'NONE',  ( 9.199394841453944593, -282.7656273979195021, -331.6772722200328758 ) ) ;
#16244=CARTESIAN_POINT ( 'NONE',  ( 18.84965566818484817, -281.2240649149354113, -223.7089026532827063 ) ) ;
#16245=CARTESIAN_POINT ( 'NONE',  ( -112.3417001280813707, -270.0523547857347353, -270.3292895737510548 ) ) ;
#16246=CARTESIAN_POINT ( 'NONE',  ( 190.2525334769776180, 271.2110853878423882, -139.6778337214551300 ) ) ;
#16248=CARTESIAN_POINT ( 'NONE',  ( -6.735091568210989976, -278.6495834679942050, -338.6492131537686419 ) ) ;
#16249=CARTESIAN_POINT ( 'NONE',  ( -49.07113805792994299, -154.4069795088023511, -364.5415411693985561 ) ) ;
#16250=CARTESIAN_POINT ( 'NONE',  ( -65.60447484896799608, -297.0210948122020227, -202.9437001037192090 ) ) ;
#16251=CARTESIAN_POINT ( 'NONE',  ( 34.40771299638171143, -292.7059853519118064, -242.4370930409610594 ) ) ;
#16252=CARTESIAN_POINT ( 'NONE',  ( -54.76359932913371864, -169.9329552033845516, -360.8268486737666194 ) ) ;
#16253=CARTESIAN_POINT ( 'NONE',  ( -57.21880872032244980, -296.3754306481411049, -196.5261409564130304 ) ) ;
#16254=CARTESIAN_POINT ( 'NONE',  ( -34.56812770239302779, -287.4167306199391305, -344.1591099195398442 ) ) ;
#16255=CARTESIAN_POINT ( 'NONE',  ( -31.48160652108500912, -296.8379384946323967, -344.4156246562875481 ) ) ;
#16256=CARTESIAN_POINT ( 'NONE',  ( -60.14745262134368176, -287.0654195245782603, -200.4959540560353446 ) ) ;
#16258=CARTESIAN_POINT ( 'NONE',  ( 11.05927667204722020, -295.3424024451439323, -330.0128941925360664 ) ) ;
#16259=CARTESIAN_POINT ( 'NONE',  ( -92.60156605940046859, -284.3638789883883078, -318.1748787456050991 ) ) ;
#16260=CARTESIAN_POINT ( 'NONE',  ( -23.43396497331633910, -297.0175644046451566, -193.7609613474342041 ) ) ;
#16261=CARTESIAN_POINT ( 'NONE',  ( -22.23556206878428299, -293.0435875689218506, -194.9679170069993859 ) ) ;
#16262=CARTESIAN_POINT ( 'NONE',  ( 26.46421620400243668, -294.6113789652583250, -313.3533491906871404 ) ) ;
#16263=CARTESIAN_POINT ( 'NONE',  ( -99.71270950028346647, -291.2412504672337263, -232.4288468353344115 ) ) ;
#16266=CARTESIAN_POINT ( 'NONE',  ( -112.1228431768507505, -274.6147742318615883, -259.1824232462478790 ) ) ;
#16267=CARTESIAN_POINT ( 'NONE',  ( 37.25179132366939427, -274.1273084720768907, -252.8735815603266417 ) ) ;
#16268=ADVANCED_FACE ( 'NONE', ( #2218 ), #22578, .F. ) ;
#16270=CARTESIAN_POINT ( 'NONE',  ( 16.90738480389926579, -275.8124252127422551, -324.9933978776310823 ) ) ;
#16271=CARTESIAN_POINT ( 'NONE',  ( -44.61846469467364784, -296.4384195630203180, -196.9770698065047725 ) ) ;
#16272=CARTESIAN_POINT ( 'NONE',  ( -110.1025740669333999, -280.6043674298349515, -255.5757484245055764 ) ) ;
#16273=CARTESIAN_POINT ( 'NONE',  ( -54.25804351974434070, -275.4111532736019399, -342.6962504152160705 ) ) ;
#16274=CARTESIAN_POINT ( 'NONE',  ( -107.8450367566909023, -298.0256707143407198, -249.9549907261361170 ) ) ;
#16275=CARTESIAN_POINT ( 'NONE',  ( -108.7670278209491102, -273.7061770371675493, -254.1799247962115942 ) ) ;
#16276=CARTESIAN_POINT ( 'NONE',  ( -89.48402620175262712, -275.0901107349373547, -215.0158144447745485 ) ) ;
#16277=CARTESIAN_POINT ( 'NONE',  ( -43.87448814499236249, -271.9902098740429892, -195.2374532410689483 ) ) ;
#16278=CARTESIAN_POINT ( 'NONE',  ( -95.68067244368005220, -296.5853736950767825, -314.4323543006391901 ) ) ;
#16279=CARTESIAN_POINT ( 'NONE',  ( -19.91516919216364556, -290.8551404308154247, -198.8123333606396557 ) ) ;
#16281=CARTESIAN_POINT ( 'NONE',  ( -38.53771001915254857, -277.5591169839955796, -347.2902832181782173 ) ) ;
#16282=CARTESIAN_POINT ( 'NONE',  ( 32.06115075511849710, -275.4165693455886412, -247.5657063917959704 ) ) ;
#16283=CARTESIAN_POINT ( 'NONE',  ( -87.41445348585385489, -284.0558691444924193, -212.4462236600289771 ) ) ;
#16284=CARTESIAN_POINT ( 'NONE',  ( -100.0835885964505110, -297.9936164148354010, -311.8494529010843053 ) ) ;
#16286=CARTESIAN_POINT ( 'NONE',  ( -85.82552796069502676, -284.5577152500976013, -215.5036335218603369 ) ) ;
#16287=CARTESIAN_POINT ( 'NONE',  ( -110.4423378051600508, -282.3270707865679015, -287.9178278497233805 ) ) ;
#16288=CARTESIAN_POINT ( 'NONE',  ( -100.0453493371967397, -276.2553354315428464, -309.7789801721383469 ) ) ;
#16289=CARTESIAN_POINT ( 'NONE',  ( -83.38948806981899509, -276.2719699245692482, -327.8285966362729482 ) ) ;
#16290=CARTESIAN_POINT ( 'NONE',  ( -81.50644578307097277, -281.4518903907718368, -209.6801187859854281 ) ) ;
#16291=CARTESIAN_POINT ( 'NONE',  ( 22.59627237185681992, -276.1688468478930645, -227.9770027233890914 ) ) ;
#16293=CARTESIAN_POINT ( 'NONE',  ( -107.3345166760472438, -271.3413186390429246, -240.1039143176219000 ) ) ;
#16294=CARTESIAN_POINT ( 'NONE',  ( -100.3682369741816416, -281.1044126406736723, -229.3073459555960767 ) ) ;
#16296=CARTESIAN_POINT ( 'NONE',  ( 4.364098886497129293, -288.5295649036525560, -207.2913468105184904 ) ) ;
#16298=CARTESIAN_POINT ( 'NONE',  ( -79.68695810032636473, -287.6238753389943099, -332.3254821489668984 ) ) ;
#16300=CARTESIAN_POINT ( 'NONE',  ( -88.39095327756177767, -296.1125388482879544, -217.5539986676623414 ) ) ;
#16301=CARTESIAN_POINT ( 'NONE',  ( -111.5724348540797735, -288.6811625316134950, -271.1756727572679324 ) ) ;
#16302=CARTESIAN_POINT ( 'NONE',  ( -47.20788896421541381, -156.8319029772612225, -362.3615984655540387 ) ) ;
#16304=CARTESIAN_POINT ( 'NONE',  ( 38.88616731575952912, -285.9754619152517421, -265.8785973540325926 ) ) ;
#16305=CARTESIAN_POINT ( 'NONE',  ( -59.16547274837295589, -284.9393466231269940, -340.9142227803303626 ) ) ;
#16306=CARTESIAN_POINT ( 'NONE',  ( -109.2727562147464937, -282.4793054143922291, -294.8539165807092672 ) ) ;
#16307=CARTESIAN_POINT ( 'NONE',  ( -91.67315886739584130, -291.2500997714784035, -221.5869846503155713 ) ) ;
#16308=CARTESIAN_POINT ( 'NONE',  ( 18.39906502073738537, -282.2984139532649692, -222.2965724808200321 ) ) ;
#16309=CARTESIAN_POINT ( 'NONE',  ( 33.91534250338784062, -282.1366924023305387, -253.7769205953290736 ) ) ;
#16310=CARTESIAN_POINT ( 'NONE',  ( -110.9530855807429361, -292.3260695792760089, -286.4785228289846941 ) ) ;
#16311=CARTESIAN_POINT ( 'NONE',  ( -54.59722990014531518, -298.0029883143106986, -195.3194848928578438 ) ) ;
#16312=CARTESIAN_POINT ( 'NONE',  ( -38.91516943878473711, -287.1515998151572262, -345.9047371424738913 ) ) ;
#16313=CARTESIAN_POINT ( 'NONE',  ( 22.64100153086099709, -276.1994314979034471, -318.6631865093805800 ) ) ;
#16314=CARTESIAN_POINT ( 'NONE',  ( -64.69735070395229570, -293.6731113546075562, -200.8957466590317154 ) ) ;
#16316=CARTESIAN_POINT ( 'NONE',  ( 31.95455697924148097, -289.6233781216988064, -236.9535640164627637 ) ) ;
#16317=CARTESIAN_POINT ( 'NONE',  ( -70.77876011418413782, -275.4920321172583613, -337.6811852012679651 ) ) ;
#16319=CARTESIAN_POINT ( 'NONE',  ( -97.58878990773281714, -295.5816866356868218, -223.6846435349226283 ) ) ;
#16320=CARTESIAN_POINT ( 'NONE',  ( -96.35875916494275373, -272.5049752317430602, -227.1391175805158014 ) ) ;
#16321=CARTESIAN_POINT ( 'NONE',  ( -104.6733955762617825, -291.6713406214026350, -300.4395371104528749 ) ) ;
#16323=CARTESIAN_POINT ( 'NONE',  ( -34.86128085730018711, -293.0253279964703097, -197.1678398149136910 ) ) ;
#16324=CARTESIAN_POINT ( 'NONE',  ( -86.41455260513905046, -287.1202765448499008, -214.8865596164082206 ) ) ;
#16326=CARTESIAN_POINT ( 'NONE',  ( -2.342030346994991685, -293.9312962688777020, -202.4227520566249723 ) ) ;
#16327=CARTESIAN_POINT ( 'NONE',  ( 20.92392625531129369, -294.1942918371789801, -220.7587026231051652 ) ) ;
#16328=CARTESIAN_POINT ( 'NONE',  ( 35.29555480958364200, -293.2831422041878113, -262.6040241040332717 ) ) ;
#16329=CARTESIAN_POINT ( 'NONE',  ( 37.11265630975704255, -289.6682648502039683, -279.3915916932880918 ) ) ;
#16330=CARTESIAN_POINT ( 'NONE',  ( 38.87156924947326786, -281.8561386452170154, -281.3400785568035758 ) ) ;
#16331=CARTESIAN_POINT ( 'NONE',  ( -34.09893422739740743, -296.1722966420492753, -194.8021611526462777 ) ) ;
#16332=CARTESIAN_POINT ( 'NONE',  ( -113.9040879143121003, -284.2829502187655635, -278.5587262293210529 ) ) ;
#16333=CARTESIAN_POINT ( 'NONE',  ( -0.6400002919494620635, -278.5422975026340282, -335.4183253151110193 ) ) ;
#16335=CARTESIAN_POINT ( 'NONE',  ( -44.04544713944608958, -284.7604256844923043, -197.2708294291886943 ) ) ;
#16336=CARTESIAN_POINT ( 'NONE',  ( 35.86699938998306436, -285.7619569205180028, -286.7134317703620923 ) ) ;
#16337=CARTESIAN_POINT ( 'NONE',  ( -61.62888077925511965, -277.8796278114597271, -198.5392395433031254 ) ) ;
#16338=CARTESIAN_POINT ( 'NONE',  ( -91.56268290671289378, -284.7612444521975021, -221.3166591200748883 ) ) ;
#16339=CARTESIAN_POINT ( 'NONE',  ( -1.335711987239448284, -281.7240120381648012, -202.7476759949971665 ) ) ;
#16340=CARTESIAN_POINT ( 'NONE',  ( -95.28858787518115037, -288.9282944163298339, -320.7096871167536278 ) ) ;
#16341=CARTESIAN_POINT ( 'NONE',  ( -17.93349189183457071, -296.5586122712506381, -341.7844717555098555 ) ) ;
#16342=CARTESIAN_POINT ( 'NONE',  ( -104.2631767810817252, -279.6757331693218589, -306.8022537521929962 ) ) ;
#16343=CARTESIAN_POINT ( 'NONE',  ( -5.474815611269156612, -277.9567955228624214, -339.9154129302462479 ) ) ;
#16344=CARTESIAN_POINT ( 'NONE',  ( -99.17622246392538443, -277.8485398082911502, -309.2562126029421847 ) ) ;
#16345=CARTESIAN_POINT ( 'NONE',  ( -39.23973409271948043, -300.0284663701080490, -195.5391343674373559 ) ) ;
#16346=CARTESIAN_POINT ( 'NONE',  ( 18.26968700832773607, -284.8524379816008718, -220.2680141096455770 ) ) ;
#16347=CARTESIAN_POINT ( 'NONE',  ( -62.48029895242832055, -290.9738467421628343, -342.3508475376461320 ) ) ;
#16348=CARTESIAN_POINT ( 'NONE',  ( -67.43461775610808218, -294.3767146558628269, -337.2227883698180904 ) ) ;
#16350=CARTESIAN_POINT ( 'NONE',  ( -13.00519557605837306, -294.3938750924319834, -339.2607555079485451 ) ) ;
#16351=CARTESIAN_POINT ( 'NONE',  ( -108.5064889487205875, -291.2675865707088292, -298.9454728142289355 ) ) ;
#16352=CARTESIAN_POINT ( 'NONE',  ( -110.3816463245337332, -279.1639205000208790, -273.3709232058374710 ) ) ;
#16353=CARTESIAN_POINT ( 'NONE',  ( -95.84057788451019633, -272.2832339461539277, -220.6347312962411138 ) ) ;
#16354=CARTESIAN_POINT ( 'NONE',  ( 39.47532038430919243, -288.1466475145248296, -265.8161411878350577 ) ) ;
#16355=CARTESIAN_POINT ( 'NONE',  ( -6.924373560759228496, -288.9970583541010569, -341.0897840895344189 ) ) ;
#16357=CARTESIAN_POINT ( 'NONE',  ( -94.14116556072769981, -285.5344308015914976, -224.4511234692889161 ) ) ;
#16359=CARTESIAN_POINT ( 'NONE',  ( 101.6393219532830017, 116.6108303934152559, -281.7644831123793665 ) ) ;
#16360=CARTESIAN_POINT ( 'NONE',  ( -107.7063693688264578, -264.2743598394135915, -305.3713782035580948 ) ) ;
#16361=CARTESIAN_POINT ( 'NONE',  ( 13.83699699917069914, -275.5094207430456663, -322.7130432056569020 ) ) ;
#16362=CARTESIAN_POINT ( 'NONE',  ( -108.9055166516405677, -277.6820436282390574, -254.4025626319421747 ) ) ;
#16363=CARTESIAN_POINT ( 'NONE',  ( -106.8223142620483515, -272.6438231725377932, -237.2221899521937303 ) ) ;
#16364=CARTESIAN_POINT ( 'NONE',  ( 7.303344965765894869, -59.94948904379861432, -351.8522816994340587 ) ) ;
#16365=CARTESIAN_POINT ( 'NONE',  ( -105.9108815046298275, -276.7966955586236963, -304.4150898271585106 ) ) ;
#16366=CARTESIAN_POINT ( 'NONE',  ( -58.54675827214202855, -297.0826488908067518, -343.3838887269895963 ) ) ;
#16367=CARTESIAN_POINT ( 'NONE',  ( -89.86491333119911928, -291.7777575810740132, -219.5743035867909327 ) ) ;
#16368=CARTESIAN_POINT ( 'NONE',  ( -98.11256362570412648, -297.9842581717509233, -223.3179591224055400 ) ) ;
#16369=CARTESIAN_POINT ( 'NONE',  ( -114.2400753769498323, -273.2393221503794507, -267.5057244075153449 ) ) ;
#16370=CARTESIAN_POINT ( 'NONE',  ( -92.74579171207487605, -297.3956677056554554, -222.8088843005247384 ) ) ;
#16373=CARTESIAN_POINT ( 'NONE',  ( -110.4282333791863238, -280.2271201044817985, -289.5866907514853210 ) ) ;
#16374=CARTESIAN_POINT ( 'NONE',  ( -33.06843756209846674, -282.5073680209209783, -347.1939413502580010 ) ) ;
#16376=CARTESIAN_POINT ( 'NONE',  ( -102.4366631083095314, -280.0897522725324507, -236.5330680631435314 ) ) ;
#16377=CARTESIAN_POINT ( 'NONE',  ( -73.59341721139551851, -279.2865404823958784, -337.1575573643905841 ) ) ;
#16378=CARTESIAN_POINT ( 'NONE',  ( -3.771726761362441227, -272.9832408635779188, -204.7438661822537824 ) ) ;
#16380=CARTESIAN_POINT ( 'NONE',  ( 202.9738562182569694, 295.9636489450776367, -54.00000000004089173 ) ) ;
#16381=CARTESIAN_POINT ( 'NONE',  ( -39.70335924761886304, -280.1883842873778576, -197.3868097963167543 ) ) ;
#16382=CARTESIAN_POINT ( 'NONE',  ( 26.00564014826802861, -275.7795570244337569, -226.8490291283033855 ) ) ;
#16383=CARTESIAN_POINT ( 'NONE',  ( 35.98450153386072969, -277.3492191523527026, -254.5439510777742100 ) ) ;
#16384=CARTESIAN_POINT ( 'NONE',  ( 5.525604941588728281, -275.0586695930691121, -333.6145799252662414 ) ) ;
#16387=CARTESIAN_POINT ( 'NONE',  ( 37.54518467823262995, -283.4190283348060007, -261.5174182045536782 ) ) ;
#16388=CARTESIAN_POINT ( 'NONE',  ( -108.5823706773655033, -289.9692508772018300, -253.6521297974555011 ) ) ;
#16389=CARTESIAN_POINT ( 'NONE',  ( -64.50341495112634504, -285.0553511108719817, -198.4056462179503910 ) ) ;
#16390=CARTESIAN_POINT ( 'NONE',  ( -109.4171676094219237, -282.5724361356600980, -287.2421713934564309 ) ) ;
#16391=CARTESIAN_POINT ( 'NONE',  ( 3.703943885315436280, -281.0629207807710372, -331.5016306394239223 ) ) ;
#16392=CARTESIAN_POINT ( 'NONE',  ( 34.05796650964800421, -285.3582323336006539, -249.2589922416829040 ) ) ;
#16393=CARTESIAN_POINT ( 'NONE',  ( -19.45255041007359154, -281.4923699012830980, -199.1249191239672598 ) ) ;
#16394=CARTESIAN_POINT ( 'NONE',  ( -112.3407539019156900, -270.5881751857016297, -267.5427233129597084 ) ) ;
#16395=CARTESIAN_POINT ( 'NONE',  ( 4.093413111189980746, -280.9041483905016889, -334.3732316026350873 ) ) ;
#16396=CARTESIAN_POINT ( 'NONE',  ( 19.85925050791570712, -296.2235695291658999, -318.8693842686535049 ) ) ;
#16397=CARTESIAN_POINT ( 'NONE',  ( -85.16567056974426464, -278.3843260780103037, -325.7161428276451716 ) ) ;
#16398=CARTESIAN_POINT ( 'NONE',  ( -75.20577320404669308, -287.5493480377762694, -205.3678154330653740 ) ) ;
#16400=CARTESIAN_POINT ( 'NONE',  ( -97.22235877942109994, -293.0991270643964413, -224.2574108282517216 ) ) ;
#16401=CARTESIAN_POINT ( 'NONE',  ( 36.11849887208956034, -273.7461268645795371, -285.4806356723203180 ) ) ;
#16402=CARTESIAN_POINT ( 'NONE',  ( -4.411556307768401020, -287.8263332408782844, -339.8000893942184462 ) ) ;
#16403=CARTESIAN_POINT ( 'NONE',  ( 4.978900444463637776, -291.0342278158880163, -209.8384981112743333 ) ) ;
#16405=CARTESIAN_POINT ( 'NONE',  ( -83.32829433658616836, -276.3820504910677869, -327.7544270997032640 ) ) ;
#16406=CARTESIAN_POINT ( 'NONE',  ( -84.84740977078065782, -295.5289858015545406, -213.2495379198569765 ) ) ;
#16407=CARTESIAN_POINT ( 'NONE',  ( -108.1967933285187229, -291.6090009648519867, -290.0625747719290075 ) ) ;
#16410=CARTESIAN_POINT ( 'NONE',  ( 25.13574854362705935, -292.6168872873300302, -314.1934580407796034 ) ) ;
#16411=CARTESIAN_POINT ( 'NONE',  ( 33.03035483248249449, -288.8602792956152712, -248.0879171870295181 ) ) ;
#16412=CARTESIAN_POINT ( 'NONE',  ( -112.8099185932005639, -288.6741950223462254, -279.6577538929920479 ) ) ;
#16413=CARTESIAN_POINT ( 'NONE',  ( 35.34405464604518698, -289.1289174953184897, -281.9374564280342952 ) ) ;
#16415=CARTESIAN_POINT ( 'NONE',  ( 34.68245126903803310, -288.5241268484272155, -283.2111507764303724 ) ) ;
#16416=CARTESIAN_POINT ( 'NONE',  ( -67.54331271831900096, -297.4262855566577741, -339.3992914978597355 ) ) ;
#16419=CARTESIAN_POINT ( 'NONE',  ( -36.07792257828234028, -290.2417407020392375, -346.9666639826853611 ) ) ;
#16420=CARTESIAN_POINT ( 'NONE',  ( -8.150367190403326134, -278.4526473076394950, -200.8757362775862418 ) ) ;
#16421=CARTESIAN_POINT ( 'NONE',  ( -110.6452279083395780, -278.5879157333712328, -294.0345653154408865 ) ) ;
#16422=CARTESIAN_POINT ( 'NONE',  ( -91.04037723865688747, -278.9815942206272439, -215.1307013957088259 ) ) ;
#16423=CARTESIAN_POINT ( 'NONE',  ( -85.14714502091128168, -299.3686759873275491, -212.9657288373902873 ) ) ;
#16424=CARTESIAN_POINT ( 'NONE',  ( -109.9589137582513132, -282.7929746611975474, -251.6063602795169345 ) ) ;
#16425=CARTESIAN_POINT ( 'NONE',  ( -110.4232819666299292, -271.9154740667189003, -270.3530115452461473 ) ) ;
#16426=CARTESIAN_POINT ( 'NONE',  ( -30.11901669293905570, -278.2839448855958722, -196.4269062987093548 ) ) ;
#16427=CARTESIAN_POINT ( 'NONE',  ( -102.6873169358189699, -282.0604138633944444, -307.2760261478925372 ) ) ;
#16428=CARTESIAN_POINT ( 'NONE',  ( -93.16753622582476169, -239.2408764263383887, -338.7286017555671265 ) ) ;
#16429=CARTESIAN_POINT ( 'NONE',  ( 21.18627014143743281, -274.6969471670539633, -319.3221683276909744 ) ) ;
#16430=CARTESIAN_POINT ( 'NONE',  ( -93.59926889214534640, -297.4019141856183523, -317.9810143550502630 ) ) ;
#16431=CARTESIAN_POINT ( 'NONE',  ( 36.88913658842953680, -280.7146235228121895, -289.6296257362170081 ) ) ;
#16432=CARTESIAN_POINT ( 'NONE',  ( -108.5248874333462226, -297.2663434550825627, -287.6291426650424796 ) ) ;
#16433=CARTESIAN_POINT ( 'NONE',  ( 98.08324619808344380, -301.0295057411529456, -193.8246312193383289 ) ) ;
#16434=CARTESIAN_POINT ( 'NONE',  ( -32.68544533119239048, -273.7791351950536978, -197.4760501967423920 ) ) ;
#16435=CARTESIAN_POINT ( 'NONE',  ( 26.13315106313796221, -296.0905427342914891, -310.4079913028380702 ) ) ;
#16436=CARTESIAN_POINT ( 'NONE',  ( 16.29766802551027993, -286.9554033782414990, -215.1178542431868550 ) ) ;
#16437=CARTESIAN_POINT ( 'NONE',  ( -33.95488338532514661, -278.1742984622959511, -194.8770556098618272 ) ) ;
#16438=CARTESIAN_POINT ( 'NONE',  ( -93.59424724881260715, -289.6677639854623862, -323.0179119074566074 ) ) ;
#16439=CARTESIAN_POINT ( 'NONE',  ( -70.08840475228363687, -288.5532730354867113, -335.8812196734693885 ) ) ;
#16440=CARTESIAN_POINT ( 'NONE',  ( -19.82841323456613125, -290.2769892473327786, -197.3811393204888702 ) ) ;
#16443=CARTESIAN_POINT ( 'NONE',  ( -108.4859596646804931, -290.2796859565485192, -253.6788072434247852 ) ) ;
#16445=CARTESIAN_POINT ( 'NONE',  ( 20.10267974825305970, -287.8007702458906465, -219.3615160238268231 ) ) ;
#16446=CARTESIAN_POINT ( 'NONE',  ( 27.33386217378599881, -289.6233781216987495, -239.1787733560258573 ) ) ;
#16447=CARTESIAN_POINT ( 'NONE',  ( -39.11445639276230679, -294.1326430087868857, -347.1053526129744569 ) ) ;
#16448=CARTESIAN_POINT ( 'NONE',  ( -16.26153551749690607, -284.1005004927590107, -343.9614473518827253 ) ) ;
#16449=CARTESIAN_POINT ( 'NONE',  ( -54.75428191579339199, -285.6554974714052832, -199.4159294301886405 ) ) ;
#16450=CARTESIAN_POINT ( 'NONE',  ( 33.72330486385948234, -277.1130583691019638, -289.0963400157307319 ) ) ;
#16451=CARTESIAN_POINT ( 'NONE',  ( 12.03735191561217910, -290.7623452765506613, -214.3139498349991641 ) ) ;
#16452=CARTESIAN_POINT ( 'NONE',  ( 0.8320156675063714591, -273.3686904842926992, -207.6722200255360349 ) ) ;
#16454=CARTESIAN_POINT ( 'NONE',  ( -114.4693268140674434, -273.6886850827510216, -284.2063049943780015 ) ) ;
#16455=CARTESIAN_POINT ( 'NONE',  ( -3.970510213944848932, -288.4159819672958065, -203.8203193325850862 ) ) ;
#16456=CARTESIAN_POINT ( 'NONE',  ( -87.27147981212841898, -298.4550727300872381, -212.0801943329517485 ) ) ;
#16457=CARTESIAN_POINT ( 'NONE',  ( -46.74619177966876293, -286.5811557660247217, -197.8158011370420297 ) ) ;
#16458=CARTESIAN_POINT ( 'NONE',  ( -103.4094153688019162, -277.0989664413390869, -309.5534556415274210 ) ) ;
#16459=CARTESIAN_POINT ( 'NONE',  ( 21.22741372987772834, -293.5306383462622648, -220.5115782348033235 ) ) ;
#16460=CARTESIAN_POINT ( 'NONE',  ( 38.36874495764529058, -285.7428343245421729, -274.3813994664754432 ) ) ;
#16461=CARTESIAN_POINT ( 'NONE',  ( -30.58857772933567531, -295.3022437969684688, -347.0431864821463819 ) ) ;
#16462=CARTESIAN_POINT ( 'NONE',  ( -96.78104473609431579, -291.4788819079716973, -227.8603537622912540 ) ) ;
#16465=FACE_OUTER_BOUND ( 'NONE', #40184, .T. ) ;
#16466=CARTESIAN_POINT ( 'NONE',  ( -93.42344398682644169, -286.7838328139675355, -218.5386496676854335 ) ) ;
#16467=CARTESIAN_POINT ( 'NONE',  ( -19.05039376806006857, -271.7666405000204009, -190.3683826091709363 ) ) ;
#16469=CARTESIAN_POINT ( 'NONE',  ( -90.97695450167036313, -282.7568732130407057, -320.3359672776710454 ) ) ;
#16470=CARTESIAN_POINT ( 'NONE',  ( -97.67767780035426028, -278.8587599411739575, -222.5561591393152696 ) ) ;
#16471=CARTESIAN_POINT ( 'NONE',  ( 28.47939625975084610, -284.0261726326654639, -305.9646528356768158 ) ) ;
#16472=CARTESIAN_POINT ( 'NONE',  ( -20.11176207632858137, -109.5359415251419506, -361.5385522582666340 ) ) ;
#16473=CARTESIAN_POINT ( 'NONE',  ( -35.92843382695069465, -281.6095211396936406, -346.7718374575732128 ) ) ;
#16474=CARTESIAN_POINT ( 'NONE',  ( -3.834117088620982994, -284.5165667996649290, -203.6596286045912052 ) ) ;
#16475=CARTESIAN_POINT ( 'NONE',  ( -34.17885669190302167, -275.9519435702060832, -194.6623603719603182 ) ) ;
#16476=CARTESIAN_POINT ( 'NONE',  ( -93.66502482366470872, -297.7038360009959206, -223.8048774715532545 ) ) ;
#16477=CARTESIAN_POINT ( 'NONE',  ( -34.29741842752031999, -293.6979010685468552, -343.7911923928651277 ) ) ;
#16478=CARTESIAN_POINT ( 'NONE',  ( -114.2827779164243935, -279.1878616153184112, -271.6150246088460563 ) ) ;
#16479=CARTESIAN_POINT ( 'NONE',  ( 20.02246176103595587, -276.1892285223080989, -315.5293710900151041 ) ) ;
#16480=CARTESIAN_POINT ( 'NONE',  ( -93.92652099347314731, -274.3388772928976209, -218.5763831155590537 ) ) ;
#16481=CARTESIAN_POINT ( 'NONE',  ( 8.047007390352755252, -275.3685137908680076, -332.2439903706264204 ) ) ;
#16482=CARTESIAN_POINT ( 'NONE',  ( 202.9738562182569694, 295.9636489450776367, -54.00000000004089173 ) ) ;
#16483=CARTESIAN_POINT ( 'NONE',  ( -39.18398525744974137, -275.0750839925356672, -345.3511302715397733 ) ) ;
#16484=CARTESIAN_POINT ( 'NONE',  ( -36.26440983036671639, -296.4641969178428553, -346.7773000663530070 ) ) ;
#16488=CARTESIAN_POINT ( 'NONE',  ( -110.6271891850301330, -285.5884205087698433, -273.6657232316608770 ) ) ;
#16489=CARTESIAN_POINT ( 'NONE',  ( -49.90361924240939118, -284.9702995300782504, -345.3554070977949095 ) ) ;
#16490=CARTESIAN_POINT ( 'NONE',  ( -4.541398034956920959, -285.8448308217389240, -205.0309346739786349 ) ) ;
#16491=CARTESIAN_POINT ( 'NONE',  ( -85.99648656322791851, -277.7642414396756294, -214.8710092223476522 ) ) ;
#16492=CARTESIAN_POINT ( 'NONE',  ( -110.6445316755044246, -286.5657634965576221, -258.5518267821323661 ) ) ;
#16493=CARTESIAN_POINT ( 'NONE',  ( -49.23491877125587024, -278.3776952845079222, -197.6338252979622609 ) ) ;
#16495=CARTESIAN_POINT ( 'NONE',  ( -66.91480399848555294, -278.5287697493715768, -337.4406051737995540 ) ) ;
#16498=CARTESIAN_POINT ( 'NONE',  ( -40.78411110627732228, -274.5001739641683685, -197.3309793621284882 ) ) ;
#16499=CARTESIAN_POINT ( 'NONE',  ( 37.39371018297305937, -282.5793987640058162, -288.2716080552581275 ) ) ;
#16500=CARTESIAN_POINT ( 'NONE',  ( 37.27004240184719208, -281.8093584697490428, -251.5830781455788951 ) ) ;
#16504=CARTESIAN_POINT ( 'NONE',  ( 23.69391603993715378, -288.8065495477807758, -225.4728228318831214 ) ) ;
#16505=CARTESIAN_POINT ( 'NONE',  ( -110.2101549340380018, -295.8426013340413760, -263.2738676620968477 ) ) ;
#16506=CARTESIAN_POINT ( 'NONE',  ( -39.20090162447199589, -291.3780169100749049, -193.4725110917958091 ) ) ;
#16507=CARTESIAN_POINT ( 'NONE',  ( 33.70278637241463571, -285.7757349934631748, -250.7808041061944664 ) ) ;
#16508=CARTESIAN_POINT ( 'NONE',  ( 21.63491651461685450, -286.7397549024686896, -314.3950853371051153 ) ) ;
#16509=CARTESIAN_POINT ( 'NONE',  ( -22.51603766146757124, -290.4844075091629065, -197.8478520005486985 ) ) ;
#16510=CARTESIAN_POINT ( 'NONE',  ( -2.008638853555458681, -287.7357984502024237, -205.9713285316565532 ) ) ;
#16511=CARTESIAN_POINT ( 'NONE',  ( -112.0882334939014982, -276.4651448873058257, -277.1246959048369263 ) ) ;
#16512=CARTESIAN_POINT ( 'NONE',  ( -54.34315832023415282, -287.6667457335944960, -344.6944057267452308 ) ) ;
#16513=CARTESIAN_POINT ( 'NONE',  ( -16.00740602988867778, -288.3280766878202712, -198.4055119750116774 ) ) ;
#16514=CARTESIAN_POINT ( 'NONE',  ( -98.39638342483668509, -287.9564642696454371, -314.2278384150113766 ) ) ;
#16515=CARTESIAN_POINT ( 'NONE',  ( -53.73070220970032551, -284.2087921836017017, -341.7912992270585164 ) ) ;
#16516=CARTESIAN_POINT ( 'NONE',  ( -87.44682410682791840, -293.3551532500932240, -214.3298323020380280 ) ) ;
#16519=CARTESIAN_POINT ( 'NONE',  ( -110.2394469566807516, -298.7282720623109071, -250.2870842909765088 ) ) ;
#16520=CARTESIAN_POINT ( 'NONE',  ( -16.86675146023991800, -279.5206228940199935, -200.1231068804207496 ) ) ;
#16521=CARTESIAN_POINT ( 'NONE',  ( 26.86120017710582886, -279.0314419258011753, -231.4920272185184444 ) ) ;
#16522=CARTESIAN_POINT ( 'NONE',  ( -30.61529171246746017, -294.1663133068984735, -346.9046627805101366 ) ) ;
#16523=CARTESIAN_POINT ( 'NONE',  ( -65.86327945056973476, -296.0725328974735362, -202.2952680342497729 ) ) ;
#16524=CARTESIAN_POINT ( 'NONE',  ( 37.03950442556730849, -273.6844341870293533, -274.4149561970679656 ) ) ;
#16525=CARTESIAN_POINT ( 'NONE',  ( -103.2027118377443173, -297.4268339773159937, -303.0884990067556828 ) ) ;
#16526=CARTESIAN_POINT ( 'NONE',  ( -112.4854464783379626, -271.3050811119263699, -256.2217232971853491 ) ) ;
#16527=CARTESIAN_POINT ( 'NONE',  ( -76.57844423901413222, -293.8089776510904585, -335.4950088749483257 ) ) ;
#16528=CARTESIAN_POINT ( 'NONE',  ( -4.586988783727667496, -293.9176255201798540, -204.4494055515882849 ) ) ;
#16529=DIRECTION ( 'NONE',  ( 0.9951408606192333473, 1.205805641958531838E-17, 0.09846150276129089773 ) ) ;
#16530=CARTESIAN_POINT ( 'NONE',  ( 24.56934635180464355, -294.8934078116631667, -309.4386580128612536 ) ) ;
#16531=DIRECTION ( 'NONE',  ( 0.000000000000000000, 0.000000000000000000, 1.000000000000000000 ) ) ;
#16532=CARTESIAN_POINT ( 'NONE',  ( -65.24437450696409257, -283.7094306740340244, -200.3483568676285813 ) ) ;
#16533=CARTESIAN_POINT ( 'NONE',  ( -5.541508154679747555, -294.6218125527207121, -336.0845001079460985 ) ) ;
#16534=CARTESIAN_POINT ( 'NONE',  ( 25.10728869895594784, -282.1496775971746160, -315.4292963384559698 ) ) ;
#16535=CARTESIAN_POINT ( 'NONE',  ( 3.031495501927004455, -282.5094396885168067, -206.4297773827819071 ) ) ;
#16536=CARTESIAN_POINT ( 'NONE',  ( -100.9766187974619669, -284.7913280814240125, -226.9502066504495019 ) ) ;
#16537=CARTESIAN_POINT ( 'NONE',  ( -95.70513171976759281, -289.1979716331697432, -223.5034035790035034 ) ) ;
#16539=CARTESIAN_POINT ( 'NONE',  ( -33.19418945550215483, -284.7901519432418809, -196.9349329425350561 ) ) ;
#16540=CARTESIAN_POINT ( 'NONE',  ( -95.23403138546342461, -288.7898973745052444, -320.6599300160514190 ) ) ;
#16542=CARTESIAN_POINT ( 'NONE',  ( 10.82893419783008149, -295.9728759983894975, -326.2720328544501740 ) ) ;
#16543=CARTESIAN_POINT ( 'NONE',  ( -109.1765605292114572, -279.6441607903888098, -296.5611266592933362 ) ) ;
#16544=CARTESIAN_POINT ( 'NONE',  ( -25.19826087222318378, -292.9183127822433903, -344.7843406239869637 ) ) ;
#16545=CARTESIAN_POINT ( 'NONE',  ( 18.50778624523281124, -281.8871264321269337, -317.4222352571952115 ) ) ;
#16546=CARTESIAN_POINT ( 'NONE',  ( -4.500606725706624900, -294.7979782817109253, -340.0208505656364082 ) ) ;
#16547=CARTESIAN_POINT ( 'NONE',  ( -36.55538718224669736, -284.1417995229576263, -194.7924098791358745 ) ) ;
#16548=CARTESIAN_POINT ( 'NONE',  ( -59.06085132000310978, -279.3333775742248122, -342.1474615160801704 ) ) ;
#16550=CARTESIAN_POINT ( 'NONE',  ( 12.50628232010619989, -293.3960107692028032, -324.0830788710815682 ) ) ;
#16551=CARTESIAN_POINT ( 'NONE',  ( -34.81716171435881790, -296.0835975648974454, -195.3619699642200658 ) ) ;
#16554=CARTESIAN_POINT ( 'NONE',  ( 8.124655973759523420, -282.6567890757721671, -211.0955899426531630 ) ) ;
#16555=CARTESIAN_POINT ( 'NONE',  ( -101.5243624944597656, -295.5837371900188373, -305.2692014740655395 ) ) ;
#16558=CARTESIAN_POINT ( 'NONE',  ( 39.58706461736021254, -273.0523547857348490, -270.3937649182068981 ) ) ;
#16559=CARTESIAN_POINT ( 'NONE',  ( -90.04465218943455795, -272.5275496901165297, -214.3728379144395149 ) ) ;
#16560=CARTESIAN_POINT ( 'NONE',  ( 38.86185206922998958, -288.7745188734546105, -262.9880217815069159 ) ) ;
#16561=CARTESIAN_POINT ( 'NONE',  ( -108.7101204244019215, -290.5879318778430616, -255.0135256976755045 ) ) ;
#16562=CARTESIAN_POINT ( 'NONE',  ( -83.89053372344525883, -280.9198625248510552, -213.1643822479373682 ) ) ;
#16563=CARTESIAN_POINT ( 'NONE',  ( -77.01123119773561143, -275.1110247544981462, -208.1295446531418634 ) ) ;
#16564=CARTESIAN_POINT ( 'NONE',  ( -99.79758790485261954, -277.8769892727284514, -231.7104296342984355 ) ) ;
#16565=CARTESIAN_POINT ( 'NONE',  ( -40.56695969248433897, -279.0928470236354428, -345.3045476445147415 ) ) ;
#16567=CARTESIAN_POINT ( 'NONE',  ( -35.52165913859401059, -273.9076877626553141, -193.3695008561130635 ) ) ;
#16568=CARTESIAN_POINT ( 'NONE',  ( -55.38459516852005038, -293.7383635643948878, -198.1408428965641519 ) ) ;
#16569=DIRECTION ( 'NONE',  ( -1.000000000000000000, 0.000000000000000000, -0.000000000000000000 ) ) ;
#16571=CARTESIAN_POINT ( 'NONE',  ( 36.56180181112865313, -291.4789319421396954, -253.6122142194242599 ) ) ;
#16572=CARTESIAN_POINT ( 'NONE',  ( -35.14269840491157026, -297.7471451163913798, -197.3401024252837033 ) ) ;
#16573=CARTESIAN_POINT ( 'NONE',  ( 104.1717476309105166, -299.5541904835127980, -195.3611179825600175 ) ) ;
#16574=CARTESIAN_POINT ( 'NONE',  ( -111.2456487715862750, -291.8317643424948642, -289.4110771189849629 ) ) ;
#16575=CARTESIAN_POINT ( 'NONE',  ( -99.86837403722181250, -286.4090924074130839, -320.2651865833026363 ) ) ;
#16576=CARTESIAN_POINT ( 'NONE',  ( 27.95493599005039087, -289.0632564934966240, -233.6986580070584694 ) ) ;
#16577=CARTESIAN_POINT ( 'NONE',  ( -43.37978663416922132, -275.1284415255420868, -344.9504599700417771 ) ) ;
#16578=CARTESIAN_POINT ( 'NONE',  ( 23.65966024366784737, -278.0567709715322167, -313.1128473509648416 ) ) ;
#16579=CARTESIAN_POINT ( 'NONE',  ( -84.72723957118482474, -289.4729267960509560, -212.9509721318022173 ) ) ;
#16580=CARTESIAN_POINT ( 'NONE',  ( -95.87847397356016188, -281.0693824707078647, -222.2394647571321968 ) ) ;
#16582=CARTESIAN_POINT ( 'NONE',  ( 19.42595148636108959, -281.5517253892375038, -316.4387056566170031 ) ) ;
#16583=CARTESIAN_POINT ( 'NONE',  ( -111.7891843422113567, -279.8637154166078744, -251.8934921609886146 ) ) ;
#16584=CARTESIAN_POINT ( 'NONE',  ( 6.684191623652922409, -281.2633642591031844, -333.1135284865397921 ) ) ;
#16585=CARTESIAN_POINT ( 'NONE',  ( -96.86432128102880768, -278.8406832494876539, -318.8572366785006125 ) ) ;
#16588=CARTESIAN_POINT ( 'NONE',  ( 38.69130997034513797, -277.1537561154045761, -276.8178297470652751 ) ) ;
#16589=CARTESIAN_POINT ( 'NONE',  ( -53.35057174420112602, -288.3376638359845288, -200.3683826091709648 ) ) ;
#16591=EDGE_LOOP ( 'NONE', ( #27881, #14423, #27408, #13486 ) ) ;
#16592=CARTESIAN_POINT ( 'NONE',  ( -98.80827511514078765, -297.9690220871698330, -313.3362364723429891 ) ) ;
#16593=CARTESIAN_POINT ( 'NONE',  ( -13.17305126566774653, -289.8103282580185009, -339.5716842676411602 ) ) ;
#16594=CARTESIAN_POINT ( 'NONE',  ( -4.361561768623137603, -274.6355004930742894, -337.3391700317607160 ) ) ;
#16595=CARTESIAN_POINT ( 'NONE',  ( -106.7959276644553483, -291.9122061246599742, -301.3138820116714669 ) ) ;
#16596=CARTESIAN_POINT ( 'NONE',  ( -12.21739217684053180, -291.7363020262033046, -201.6583328883540389 ) ) ;
#16597=CARTESIAN_POINT ( 'NONE',  ( 38.72568047040571315, -286.9142102136819403, -258.7286358004117233 ) ) ;
#16599=CARTESIAN_POINT ( 'NONE',  ( -43.01452379734985954, -281.5246725783801480, -343.9934050351565133 ) ) ;
#16600=CARTESIAN_POINT ( 'NONE',  ( -75.32794126452058947, -291.4247122553418876, -334.1562276091738113 ) ) ;
#16601=CARTESIAN_POINT ( 'NONE',  ( -107.6531208500526446, -282.7422845002179770, -292.4294633829376266 ) ) ;
#16603=CARTESIAN_POINT ( 'NONE',  ( 35.19296310955536455, -283.0223503051468583, -282.1918452448913399 ) ) ;
#16604=CARTESIAN_POINT ( 'NONE',  ( 5.436172385197808765, -289.4295337490643192, -334.1017944435105846 ) ) ;
#16605=CARTESIAN_POINT ( 'NONE',  ( -68.55526625356546333, -280.1228635531553550, -204.3027972984460803 ) ) ;
#16606=CARTESIAN_POINT ( 'NONE',  ( -69.44269181578539474, -290.4339844571298386, -200.7944607697111792 ) ) ;
#16607=CARTESIAN_POINT ( 'NONE',  ( -10.06087450454213084, -287.2021139036569366, -198.4718885790336458 ) ) ;
#16608=CARTESIAN_POINT ( 'NONE',  ( -17.73395569408640071, -289.2981579022102778, -344.7591237439553424 ) ) ;
#16609=CARTESIAN_POINT ( 'NONE',  ( -67.78243368195637686, -283.6298482048885603, -336.7114137259426343 ) ) ;
#16612=CARTESIAN_POINT ( 'NONE',  ( 8.090996660351315484, -294.5258976937257671, -209.6641808921635004 ) ) ;
#16613=CARTESIAN_POINT ( 'NONE',  ( 1.504518319981962282, -293.2291034164159669, -336.2721912929378618 ) ) ;
#16614=CARTESIAN_POINT ( 'NONE',  ( -11.18115149360161986, -275.7613903733028451, -338.7645838548054940 ) ) ;
#16615=CARTESIAN_POINT ( 'NONE',  ( -85.14656004788000132, -296.7601281949540066, -210.1281689071860797 ) ) ;
#16617=CARTESIAN_POINT ( 'NONE',  ( 20.22333621356631284, -292.6760857553618393, -316.3918166350993033 ) ) ;
#16618=CARTESIAN_POINT ( 'NONE',  ( -108.4264476208809214, -295.0609326531775309, -249.7472224644902212 ) ) ;
#16619=CARTESIAN_POINT ( 'NONE',  ( -106.0879254558679463, -292.1000972868071699, -244.5052073947672113 ) ) ;
#16620=CARTESIAN_POINT ( 'NONE',  ( 4.002002081043565695, -295.5601881082467912, -330.8997367362131854 ) ) ;
#16621=CARTESIAN_POINT ( 'NONE',  ( 10.02285351824489545, -292.4014632715156381, -328.7944964748160714 ) ) ;
#16623=CARTESIAN_POINT ( 'NONE',  ( -54.95338414395156690, -299.8260138613728714, -197.4054602042285183 ) ) ;
#16624=CARTESIAN_POINT ( 'NONE',  ( 32.05975957181172475, -288.1837494451146426, -246.9763828001674995 ) ) ;
#16625=CARTESIAN_POINT ( 'NONE',  ( -45.44709109661332036, -279.1341254417251889, -345.3310606528314679 ) ) ;
#16626=CARTESIAN_POINT ( 'NONE',  ( -4.180698034977837096, -275.4195821011981025, -339.4288288812909968 ) ) ;
#16627=CARTESIAN_POINT ( 'NONE',  ( -13.08676520435249735, -273.7078072724917206, -197.3884455754348153 ) ) ;
#16628=CARTESIAN_POINT ( 'NONE',  ( 35.16851085794340293, -279.4141466836844643, -253.5211801947434083 ) ) ;
#16629=CARTESIAN_POINT ( 'NONE',  ( -86.59380599429820791, -276.1228346574709462, -328.5737064726159815 ) ) ;
#16630=CARTESIAN_POINT ( 'NONE',  ( -101.9085013149341137, -294.7610428254607768, -305.4662694744997111 ) ) ;
#16632=CARTESIAN_POINT ( 'NONE',  ( -41.88856856187663880, -298.7962259635968962, -197.3410678961627980 ) ) ;
#16634=CARTESIAN_POINT ( 'NONE',  ( -112.7445743867030501, -288.5617275316047881, -271.1850599948281229 ) ) ;
#16635=CARTESIAN_POINT ( 'NONE',  ( -95.45830251453908488, -289.8693943026705142, -320.8731019769981572 ) ) ;
#16636=CARTESIAN_POINT ( 'NONE',  ( -90.88152259847159087, -275.2946102171149505, -217.6020824004652354 ) ) ;
#16637=CARTESIAN_POINT ( 'NONE',  ( -104.4225965765146213, -294.1120329240526985, -303.6472851570148350 ) ) ;
#16638=CARTESIAN_POINT ( 'NONE',  ( -27.40313773521852170, -282.1262361771995302, -346.6074359898632338 ) ) ;
#16640=CARTESIAN_POINT ( 'NONE',  ( -3.309959604635070107, -280.6026638383646628, -337.2097237280163995 ) ) ;
#16642=CARTESIAN_POINT ( 'NONE',  ( -104.4167981935732854, -288.9465814387197042, -300.2870565187305374 ) ) ;
#16643=CARTESIAN_POINT ( 'NONE',  ( -65.81094376173723504, -281.5681259760785338, -338.9341761079012940 ) ) ;
#16646=CARTESIAN_POINT ( 'NONE',  ( 34.66336099941894133, -291.8226894915986804, -291.3898781576239685 ) ) ;
#16647=CARTESIAN_POINT ( 'NONE',  ( -79.26526013879282573, -274.9954010433622216, -209.6928279343022439 ) ) ;
#16648=CARTESIAN_POINT ( 'NONE',  ( -96.85415627650654358, -285.1067409886590553, -318.6132130463360568 ) ) ;
#16649=CARTESIAN_POINT ( 'NONE',  ( -57.70949575392910447, -271.8711450248882215, -197.5436457669048025 ) ) ;
#16650=CARTESIAN_POINT ( 'NONE',  ( -35.93346748634294840, -286.0703032089222120, -197.3747022545168761 ) ) ;
#16651=CARTESIAN_POINT ( 'NONE',  ( -13.57809017561891451, -278.1629319208394691, -340.0614111827846386 ) ) ;
#16652=CARTESIAN_POINT ( 'NONE',  ( 16.65722802147351445, -277.0616961827885802, -319.7429250538532983 ) ) ;
#16653=CARTESIAN_POINT ( 'NONE',  ( -109.1846454337006236, -286.2743845888787746, -291.9368457786694080 ) ) ;
#16656=CARTESIAN_POINT ( 'NONE',  ( -64.26817501740804062, -295.2273115250155229, -342.4996302664839618 ) ) ;
#16657=CARTESIAN_POINT ( 'NONE',  ( -46.96127114263693869, -287.9094207338338265, -196.2868315012454445 ) ) ;
#16659=CARTESIAN_POINT ( 'NONE',  ( 25.18497378105905682, -291.6952119285918457, -320.2651865833026363 ) ) ;
#16660=CARTESIAN_POINT ( 'NONE',  ( -113.9240673415976914, -277.4212706380361624, -274.4395418132581312 ) ) ;
#16661=CARTESIAN_POINT ( 'NONE',  ( -14.09096378886128953, -290.7485566597673028, -197.7395863940748200 ) ) ;
#16662=CARTESIAN_POINT ( 'NONE',  ( -110.1806611274039653, -285.9217952942664169, -281.8769456942854390 ) ) ;
#16663=CARTESIAN_POINT ( 'NONE',  ( -111.4058787188907900, -280.3083569482387247, -270.6642684498999643 ) ) ;
#16664=CARTESIAN_POINT ( 'NONE',  ( -57.61719115473270847, -287.2207739247929794, -196.6345448348295122 ) ) ;
#16665=CARTESIAN_POINT ( 'NONE',  ( 32.19820235310088918, -283.9184661564850671, -298.4538681008904746 ) ) ;
#16666=CARTESIAN_POINT ( 'NONE',  ( 29.09701888490610955, -276.2254497171056755, -309.2827908706128142 ) ) ;
#16667=CARTESIAN_POINT ( 'NONE',  ( -58.34395346716120656, -295.7994415028941262, -198.7318491403834742 ) ) ;
#16668=CARTESIAN_POINT ( 'NONE',  ( -62.04562041376767212, -279.5730908147767764, -197.3753562166192523 ) ) ;
#16669=CARTESIAN_POINT ( 'NONE',  ( -110.7796133457702581, -298.3148300733818132, -282.5343304283009047 ) ) ;
#16671=CARTESIAN_POINT ( 'NONE',  ( -20.25526795762937127, -282.7662352645560304, -195.3538533559490702 ) ) ;
#16673=CARTESIAN_POINT ( 'NONE',  ( -67.66103878417175110, -295.7982870827341344, -200.8715086904071825 ) ) ;
#16674=CARTESIAN_POINT ( 'NONE',  ( -29.71322858056420912, -276.4607539649181263, -343.0742634720691058 ) ) ;
#16675=CARTESIAN_POINT ( 'NONE',  ( 2.199830783842639192, -275.7744776916161982, -204.7526120442273054 ) ) ;
#16677=CARTESIAN_POINT ( 'NONE',  ( 34.36343591443964840, -280.9589614345642303, -297.7690306647259035 ) ) ;
#16678=CARTESIAN_POINT ( 'NONE',  ( -76.38451919106526589, -291.3422354525838500, -333.2390337592499350 ) ) ;
#16679=CARTESIAN_POINT ( 'NONE',  ( -70.44592109806045244, -299.1437502742176662, -201.6092575717512432 ) ) ;
#16680=CARTESIAN_POINT ( 'NONE',  ( -113.2106445988670345, -297.8914079548573568, -259.6872502846215980 ) ) ;
#16681=CARTESIAN_POINT ( 'NONE',  ( 36.00856305734165375, -295.3615418228174008, -255.5365667100240046 ) ) ;
#16682=CARTESIAN_POINT ( 'NONE',  ( 21.60986937353373349, -280.1858429268737609, -316.4560296767756427 ) ) ;
#16683=CARTESIAN_POINT ( 'NONE',  ( -13.87771831593073024, -282.2790091167194646, -199.6613498208154169 ) ) ;
#16684=CARTESIAN_POINT ( 'NONE',  ( -68.63093441433395014, -295.7175919946152476, -202.8024002807403861 ) ) ;
#16685=CARTESIAN_POINT ( 'NONE',  ( -100.3466352374932598, -286.7244256683174513, -227.4097521604752501 ) ) ;
#16686=CARTESIAN_POINT ( 'NONE',  ( -34.58007291766566027, -287.9371034895813182, -343.6679884395664999 ) ) ;
#16687=CARTESIAN_POINT ( 'NONE',  ( -88.66512920003211207, -231.2529867285488194, -347.6922890233383328 ) ) ;
#16689=CARTESIAN_POINT ( 'NONE',  ( -20.64298893186897388, -287.4166789574570657, -344.9791576148476224 ) ) ;
#16690=CARTESIAN_POINT ( 'NONE',  ( -4.581271205340105901, -286.1629113725178399, -205.1013157788832757 ) ) ;
#16692=CARTESIAN_POINT ( 'NONE',  ( -31.64547412384881397, -284.0615321495145054, -346.8533855063180340 ) ) ;
#16693=CARTESIAN_POINT ( 'NONE',  ( -11.48670431295657401, -274.7315812325054480, -202.0164529802044342 ) ) ;
#16694=CARTESIAN_POINT ( 'NONE',  ( -106.9739778131460355, -289.8866986808618549, -238.0968387838896945 ) ) ;
#16695=CARTESIAN_POINT ( 'NONE',  ( 29.19422860332015901, -281.7015377682966459, -231.8087772729147957 ) ) ;
#16697=CARTESIAN_POINT ( 'NONE',  ( 3.434962784590767093, -282.1094720554947912, -205.8008718855227528 ) ) ;
#16698=CARTESIAN_POINT ( 'NONE',  ( -13.42447551844505860, -283.0831286378585787, -343.5301733163346398 ) ) ;
#16699=CARTESIAN_POINT ( 'NONE',  ( -92.20843863198294343, -279.2396207305267808, -222.1898333213904380 ) ) ;
#16700=CARTESIAN_POINT ( 'NONE',  ( -4.829096099716524648, -274.1237833571632905, -337.9475929042657754 ) ) ;
#16701=CARTESIAN_POINT ( 'NONE',  ( 25.85751915286289560, -23.12262787077664328, -345.2578353262790074 ) ) ;
#16703=CARTESIAN_POINT ( 'NONE',  ( 36.83446597737987815, -277.4249723051858609, -260.4654215366804806 ) ) ;
#16704=CARTESIAN_POINT ( 'NONE',  ( -71.84640263648488201, -195.7149973669283725, -359.9635178732972918 ) ) ;
#16705=CARTESIAN_POINT ( 'NONE',  ( -79.78049287100706977, -296.8096649928742750, -210.8393443328074284 ) ) ;
#16706=CARTESIAN_POINT ( 'NONE',  ( 13.35056665728578551, -293.8731082478913095, -328.3093890327222084 ) ) ;
#16707=CARTESIAN_POINT ( 'NONE',  ( -104.8259698489561345, -260.7805594622520857, -315.6649111131378049 ) ) ;
#16708=CARTESIAN_POINT ( 'NONE',  ( -54.44549071380331640, -296.4112921872676907, -195.8891995241350799 ) ) ;
#16709=CARTESIAN_POINT ( 'NONE',  ( -96.42086381693505359, -288.3377235919174950, -314.6099530810120655 ) ) ;
#16710=CARTESIAN_POINT ( 'NONE',  ( -93.10309196270191023, -297.7246057258181509, -319.3665530137477617 ) ) ;
#16711=CARTESIAN_POINT ( 'NONE',  ( -25.07589121249525377, -287.5268792226348751, -197.8471162547541553 ) ) ;
#16713=CARTESIAN_POINT ( 'NONE',  ( 4.004675341371077835, -293.5354031762456657, -205.6197010608642302 ) ) ;
#16714=CARTESIAN_POINT ( 'NONE',  ( -100.4511374388943921, -284.5396802038633837, -307.1739875236188482 ) ) ;
#16715=CARTESIAN_POINT ( 'NONE',  ( -62.69906395948762423, -296.5242179048408957, -198.0768678473976649 ) ) ;
#16716=CARTESIAN_POINT ( 'NONE',  ( -58.90318746132933114, -292.5829258906816221, -196.6097716623713723 ) ) ;
#16717=CARTESIAN_POINT ( 'NONE',  ( 23.92242080290800388, -293.4235278237208604, -223.7966170806500656 ) ) ;
#16718=CARTESIAN_POINT ( 'NONE',  ( -98.10949659709513071, -290.1570345452356605, -310.8347689664057043 ) ) ;
#16721=CARTESIAN_POINT ( 'NONE',  ( -62.45826993683399309, -299.5892154304821702, -198.8806073488312052 ) ) ;
#16722=CARTESIAN_POINT ( 'NONE',  ( -52.45220064248928793, -272.6578244031910572, -195.2091471230187949 ) ) ;
#16724=CARTESIAN_POINT ( 'NONE',  ( -34.85050550056043051, -282.0788736089846793, -343.5665070048286225 ) ) ;
#16725=VERTEX_POINT ( 'NONE', #61393 ) ;
#16727=CARTESIAN_POINT ( 'NONE',  ( -41.38748410006525802, -276.6094357507039945, -347.2063312859026496 ) ) ;
#16728=CARTESIAN_POINT ( 'NONE',  ( -94.38387301484451086, -271.6083786179167987, -223.5158270825274656 ) ) ;
#16729=CARTESIAN_POINT ( 'NONE',  ( -95.77761551949956242, -281.0475114866662238, -224.5573629264747240 ) ) ;
#16730=CARTESIAN_POINT ( 'NONE',  ( -36.47513038266711760, -275.1807984567030871, -344.6039423210291943 ) ) ;
#16731=CARTESIAN_POINT ( 'NONE',  ( -77.74328183935186587, -298.7017095745386541, -209.0232651112983717 ) ) ;
#16732=CARTESIAN_POINT ( 'NONE',  ( -68.39321470884395637, -274.5752097577409359, -204.0208202654678757 ) ) ;
#16733=CARTESIAN_POINT ( 'NONE',  ( -95.26991934793608152, -274.9841904082319388, -221.1649092872881965 ) ) ;
#16734=CARTESIAN_POINT ( 'NONE',  ( 12.88730599588936521, -272.7688335467515799, -214.1179405367782351 ) ) ;
#16735=CARTESIAN_POINT ( 'NONE',  ( 34.16902223195484112, -294.4041884905151960, -285.5905447135049258 ) ) ;
#16736=CARTESIAN_POINT ( 'NONE',  ( 20.65842752542369709, -291.4933828295686453, -225.0487686505224474 ) ) ;
#16737=CARTESIAN_POINT ( 'NONE',  ( 144.2857639756989272, -299.5541904835127980, -201.0153591320744226 ) ) ;
#16738=CARTESIAN_POINT ( 'NONE',  ( 1.021794398023314177, -277.0471486556504601, -337.1131479218443019 ) ) ;
#16739=CARTESIAN_POINT ( 'NONE',  ( 2.928171180536085494, -274.7757281860425564, -209.4127974005153590 ) ) ;
#16741=( BOUNDED_SURFACE ( )  B_SPLINE_SURFACE ( 3, 3, ( 
 ( #25860, #40515, #17846, #75599, #81757, #83151, #76069, #18302, #82233, #83620, #24469, #46697, #45766, #60478, #39123, #47160, #74676, #89314, #18781, #11199, #76543, #17390, #46239, #68035 ),
 ( #32046, #2707, #3636, #60940, #10722, #9800, #47640, #32527, #68502, #61421, #90253, #24005, #25402, #40059, #68976, #4106, #11666, #10255, #32978, #69433, #4563, #38674, #67579, #31589 ),
 ( #75143, #63765, #48103, #91664, #19702, #92595, #92129, #26818, #28231, #57119, #27764, #56171, #78872, #62830, #56659, #20655, #41461, #49059, #77955, #85028, #27284, #85508, #55704, #70393 ),
 ( #34853, #5041, #14021, #5521, #48572, #13556, #34391, #20179, #21111, #64247, #93077, #63298, #71795, #13098, #69902, #49525, #26347, #84555, #41936, #71316, #6917, #70848, #5981, #78418 ),
 ( #62340, #42406, #55240, #12135, #12616, #84096, #19245, #91181, #6447, #77007, #35322, #77473, #85960, #40980, #49979, #33921, #42882, #1201, #93531, #80266, #8751, #746, #74090, #51837 ),
 ( #86418, #35791, #73180, #50457, #79807, #29151, #59440, #28689, #50923, #21575, #58967, #30083, #57575, #15402, #37630, #29630, #64704, #79360, #36712, #269, #14495, #43353, #86899, #65633 ),
 ( #22963, #87814, #58048, #66539, #65165, #58509, #72249, #7366, #14949, #80730, #36247, #22054, #1659, #15883, #23446, #43803, #72703, #7822, #52314, #87354, #22504, #88291, #81191, #51375 ) ),
 .UNSPECIFIED., .T., .F., .F. ) 
 B_SPLINE_SURFACE_WITH_KNOTS ( ( 4, 3, 4 ),
 ( 4, 2, 2, 2, 2, 2, 2, 2, 2, 2, 2, 4 ),
 ( 0.000000000000000000, 0.5000000000000000000, 1.000000000000000000 ),
 ( 0.000000000000000000, 0.06250000000000000000, 0.1250000000000000000, 0.2500000000000000000, 0.3750000000000000000, 0.5000000000000000000, 0.6250000000000000000, 0.7500000000000000000, 0.8125000000000000000, 0.8750000000000000000, 0.9375000000000000000, 1.000000000000000000 ),
 .UNSPECIFIED. ) 
 GEOMETRIC_REPRESENTATION_ITEM ( )  RATIONAL_B_SPLINE_SURFACE ( (
 ( 1.000000000000000000, 1.000000000000000000, 1.000000000000000000, 1.000000000000000000, 1.000000000000000000, 1.000000000000000000, 1.000000000000000000, 1.000000000000000000, 1.000000000000000000, 1.000000000000000000, 1.000000000000000000, 1.000000000000000000, 1.000000000000000000, 1.000000000000000000, 1.000000000000000000, 1.000000000000000000, 1.000000000000000000, 1.000000000000000000, 1.000000000000000000, 1.000000000000000000, 1.000000000000000000, 1.000000000000000000, 1.000000000000000000, 1.000000000000000000),
 ( 0.3333333333333333703, 0.3333333333333333703, 0.3333333333333333703, 0.3333333333333333703, 0.3333333333333333703, 0.3333333333333333703, 0.3333333333333333703, 0.3333333333333333703, 0.3333333333333333703, 0.3333333333333333703, 0.3333333333333333703, 0.3333333333333333703, 0.3333333333333333703, 0.3333333333333333703, 0.3333333333333333703, 0.3333333333333333703, 0.3333333333333333703, 0.3333333333333333703, 0.3333333333333333703, 0.3333333333333333703, 0.3333333333333333703, 0.3333333333333333703, 0.3333333333333333703, 0.3333333333333333703),
 ( 0.3333333333333333703, 0.3333333333333333703, 0.3333333333333333703, 0.3333333333333333703, 0.3333333333333333703, 0.3333333333333333703, 0.3333333333333333703, 0.3333333333333333703, 0.3333333333333333703, 0.3333333333333333703, 0.3333333333333333703, 0.3333333333333333703, 0.3333333333333333703, 0.3333333333333333703, 0.3333333333333333703, 0.3333333333333333703, 0.3333333333333333703, 0.3333333333333333703, 0.3333333333333333703, 0.3333333333333333703, 0.3333333333333333703, 0.3333333333333333703, 0.3333333333333333703, 0.3333333333333333703),
 ( 1.000000000000000000, 1.000000000000000000, 1.000000000000000000, 1.000000000000000000, 1.000000000000000000, 1.000000000000000000, 1.000000000000000000, 1.000000000000000000, 1.000000000000000000, 1.000000000000000000, 1.000000000000000000, 1.000000000000000000, 1.000000000000000000, 1.000000000000000000, 1.000000000000000000, 1.000000000000000000, 1.000000000000000000, 1.000000000000000000, 1.000000000000000000, 1.000000000000000000, 1.000000000000000000, 1.000000000000000000, 1.000000000000000000, 1.000000000000000000),
 ( 0.3333333333333333703, 0.3333333333333333703, 0.3333333333333333703, 0.3333333333333333703, 0.3333333333333333703, 0.3333333333333333703, 0.3333333333333333703, 0.3333333333333333703, 0.3333333333333333703, 0.3333333333333333703, 0.3333333333333333703, 0.3333333333333333703, 0.3333333333333333703, 0.3333333333333333703, 0.3333333333333333703, 0.3333333333333333703, 0.3333333333333333703, 0.3333333333333333703, 0.3333333333333333703, 0.3333333333333333703, 0.3333333333333333703, 0.3333333333333333703, 0.3333333333333333703, 0.3333333333333333703),
 ( 0.3333333333333333703, 0.3333333333333333703, 0.3333333333333333703, 0.3333333333333333703, 0.3333333333333333703, 0.3333333333333333703, 0.3333333333333333703, 0.3333333333333333703, 0.3333333333333333703, 0.3333333333333333703, 0.3333333333333333703, 0.3333333333333333703, 0.3333333333333333703, 0.3333333333333333703, 0.3333333333333333703, 0.3333333333333333703, 0.3333333333333333703, 0.3333333333333333703, 0.3333333333333333703, 0.3333333333333333703, 0.3333333333333333703, 0.3333333333333333703, 0.3333333333333333703, 0.3333333333333333703),
 ( 1.000000000000000000, 1.000000000000000000, 1.000000000000000000, 1.000000000000000000, 1.000000000000000000, 1.000000000000000000, 1.000000000000000000, 1.000000000000000000, 1.000000000000000000, 1.000000000000000000, 1.000000000000000000, 1.000000000000000000, 1.000000000000000000, 1.000000000000000000, 1.000000000000000000, 1.000000000000000000, 1.000000000000000000, 1.000000000000000000, 1.000000000000000000, 1.000000000000000000, 1.000000000000000000, 1.000000000000000000, 1.000000000000000000, 1.000000000000000000) ) ) 
 REPRESENTATION_ITEM ( '' )  SURFACE ( )  );
#16742=CARTESIAN_POINT ( 'NONE',  ( -96.79979644121846150, -282.5868995251412912, -318.5276663424640446 ) ) ;
#16743=CARTESIAN_POINT ( 'NONE',  ( -5.261297044893791686, -296.6311619340227708, -338.3522728317411747 ) ) ;
#16746=CARTESIAN_POINT ( 'NONE',  ( -52.11156656865038883, -285.0553676782051298, -198.7060220593892836 ) ) ;
#16747=CARTESIAN_POINT ( 'NONE',  ( -16.67104662481317945, -280.7856996581161297, -342.6836949580940654 ) ) ;
#16748=CARTESIAN_POINT ( 'NONE',  ( 3.445730556832286684, -275.0664693080626648, -331.6127335879007205 ) ) ;
#16749=CARTESIAN_POINT ( 'NONE',  ( 37.56384445359252311, -283.4922763771189125, -265.6850453032252517 ) ) ;
#16750=CARTESIAN_POINT ( 'NONE',  ( 34.50690351078471707, -276.5596619019306672, -255.3028668267381533 ) ) ;
#16753=CARTESIAN_POINT ( 'NONE',  ( -32.71064855606142174, -272.5094457136060555, -194.2889575220754068 ) ) ;
#16755=CARTESIAN_POINT ( 'NONE',  ( -105.7611832317066671, -280.9612874902786075, -239.1101099601321778 ) ) ;
#16757=CARTESIAN_POINT ( 'NONE',  ( -33.81938370745150024, -288.0163015749246256, -194.8832570773436430 ) ) ;
#16759=CARTESIAN_POINT ( 'NONE',  ( -68.88567014012960499, -287.4666953059623893, -338.4189669717387687 ) ) ;
#16761=CARTESIAN_POINT ( 'NONE',  ( -99.07554989433847936, -294.7995410783873922, -310.1539037320321768 ) ) ;
#16762=CARTESIAN_POINT ( 'NONE',  ( -95.07968986657911614, -288.0427851802686519, -317.0214868709439884 ) ) ;
#16763=CARTESIAN_POINT ( 'NONE',  ( 202.9739649223127742, 291.4636489454787807, -68.19743562414970484 ) ) ;
#16764=CARTESIAN_POINT ( 'NONE',  ( 129.8483263487583201, -299.5541904835127980, -189.0224624687345454 ) ) ;
#16765=CARTESIAN_POINT ( 'NONE',  ( 37.34888832384107360, -285.8340964401198221, -254.6765161786775877 ) ) ;
#16766=CARTESIAN_POINT ( 'NONE',  ( -76.25843857654081148, -281.8042925996973054, -335.6866834723716124 ) ) ;
#16767=CARTESIAN_POINT ( 'NONE',  ( -41.59283723867329741, -291.9972612993083771, -197.4351586069549569 ) ) ;
#16768=CARTESIAN_POINT ( 'NONE',  ( -2.889172598860140884, -281.9421060549499316, -205.3206921130092724 ) ) ;
#16769=CARTESIAN_POINT ( 'NONE',  ( 34.10030408254412038, -282.5625386368658951, -286.1294965268039618 ) ) ;
#16770=CARTESIAN_POINT ( 'NONE',  ( -98.51985169744814641, -291.9358739821950053, -314.3791311382445315 ) ) ;
#16771=CARTESIAN_POINT ( 'NONE',  ( -57.39176424503054363, -297.9671267714110741, -195.9620771260187837 ) ) ;
#16772=CARTESIAN_POINT ( 'NONE',  ( 13.61422578358280866, -286.4253054320082015, -326.2245411479219683 ) ) ;
#16773=CARTESIAN_POINT ( 'NONE',  ( 37.90567700378380778, -275.7572143237819091, -286.7577216399399163 ) ) ;
#16774=CARTESIAN_POINT ( 'NONE',  ( 19.71796841307034498, -294.8633254982221388, -222.2358540173663641 ) ) ;
#16776=CARTESIAN_POINT ( 'NONE',  ( -95.99890600148557951, -287.6948066931273615, -223.6242672951989618 ) ) ;
#16777=CARTESIAN_POINT ( 'NONE',  ( -39.92605506531148052, -275.0843633310311134, -345.4961034227234222 ) ) ;
#16779=CARTESIAN_POINT ( 'NONE',  ( -100.8713423401653984, -295.5116062250157256, -228.2609491121374958 ) ) ;
#16780=CARTESIAN_POINT ( 'NONE',  ( -91.35848012726836487, -292.8676168670893958, -220.0569634975500719 ) ) ;
#16781=CARTESIAN_POINT ( 'NONE',  ( -68.31823121472450566, -272.9828026897678797, -204.1329984060267293 ) ) ;
#16782=CARTESIAN_POINT ( 'NONE',  ( -77.65042997564236771, -293.0202398442989420, -208.6690273261512800 ) ) ;
#16783=CARTESIAN_POINT ( 'NONE',  ( -72.75119327194146024, -292.5125589461138702, -206.1981504475794509 ) ) ;
#16784=CARTESIAN_POINT ( 'NONE',  ( -111.0052614399945696, -286.4124124059106862, -262.6666796976148817 ) ) ;
#16785=CARTESIAN_POINT ( 'NONE',  ( 31.64610811718649686, -294.5516605770150704, -237.3856881399447616 ) ) ;
#16786=CARTESIAN_POINT ( 'NONE',  ( -14.03273931990282541, -293.6633895292018792, -197.4358232659970724 ) ) ;
#16787=CARTESIAN_POINT ( 'NONE',  ( -5.543426997267379086, -294.4551595132879811, -336.0854284948061945 ) ) ;
#16788=CARTESIAN_POINT ( 'NONE',  ( 12.44313600156455202, -288.7453289588218581, -214.1979508259490501 ) ) ;
#16789=CARTESIAN_POINT ( 'NONE',  ( 39.52931511702630729, -281.7850864424011661, -275.6587838214941826 ) ) ;
#16790=CARTESIAN_POINT ( 'NONE',  ( -86.50640122769459595, -295.4557300401680209, -212.9149341202095513 ) ) ;
#16791=CARTESIAN_POINT ( 'NONE',  ( -109.9765517385676219, -284.7078811437680770, -244.8037641285303323 ) ) ;
#16792=CARTESIAN_POINT ( 'NONE',  ( -8.070970862483065389, -278.6467689774736982, -339.0413441852196570 ) ) ;
#16794=CARTESIAN_POINT ( 'NONE',  ( -102.5843778676272962, -283.8016949323858853, -236.7378595884887602 ) ) ;
#16795=CARTESIAN_POINT ( 'NONE',  ( 11.10403059602818487, -286.3811501681469736, -327.6150420434058788 ) ) ;
#16796=CARTESIAN_POINT ( 'NONE',  ( -96.71393925998886232, -277.3318724533035606, -223.2947530770346702 ) ) ;
#16798=CARTESIAN_POINT ( 'NONE',  ( -80.66766575671326223, -283.1651613856255949, -329.2530483675810729 ) ) ;
#16799=CARTESIAN_POINT ( 'NONE',  ( -14.36157602354539797, -281.5485847477190191, -197.2307357035033704 ) ) ;
#16800=CARTESIAN_POINT ( 'NONE',  ( 38.74365601144216953, -286.4830707033471526, -260.1709857979043932 ) ) ;
#16801=CARTESIAN_POINT ( 'NONE',  ( -41.06812608781837781, -296.8598007078484784, -344.2933279348607698 ) ) ;
#16802=CARTESIAN_POINT ( 'NONE',  ( -31.49114240818673238, -278.5797074884438871, -346.3882651543132170 ) ) ;
#16803=CARTESIAN_POINT ( 'NONE',  ( 20.45874714393577065, -277.5491765082449547, -320.5048635039091209 ) ) ;
#16804=CARTESIAN_POINT ( 'NONE',  ( -105.2685743126416469, -278.0278963736250262, -297.0994755986157543 ) ) ;
#16805=CARTESIAN_POINT ( 'NONE',  ( -111.8320046657852771, -274.6035893181807523, -264.8158203631756464 ) ) ;
#16806=CARTESIAN_POINT ( 'NONE',  ( 5.802637724076443959, -284.6378285760636686, -209.1536450596883583 ) ) ;
#16807=CARTESIAN_POINT ( 'NONE',  ( -69.00608872204273325, -291.0617430368794203, -339.6848905027318324 ) ) ;
#16808=CARTESIAN_POINT ( 'NONE',  ( 30.86814163362985042, -292.8318591819682979, -297.3633658816049774 ) ) ;
#16810=CARTESIAN_POINT ( 'NONE',  ( 21.34092943668413866, -293.8279985027817247, -313.8172622455487613 ) ) ;
#16812=CARTESIAN_POINT ( 'NONE',  ( -89.27203257531260761, -290.8426749485843743, -326.7945573688728018 ) ) ;
#16813=CARTESIAN_POINT ( 'NONE',  ( -95.69812702311496366, -279.8213889121909688, -226.3128444855985606 ) ) ;
#16814=CARTESIAN_POINT ( 'NONE',  ( -62.72970323182380525, -296.6496020223606251, -197.9944004408036164 ) ) ;
#16815=CARTESIAN_POINT ( 'NONE',  ( 38.68353979674457577, -288.0577860275657258, -258.7203405092957951 ) ) ;
#16817=CARTESIAN_POINT ( 'NONE',  ( -4.338279829644617003, -288.9622630877383358, -339.9206767323568670 ) ) ;
#16818=CARTESIAN_POINT ( 'NONE',  ( -80.63526020985034393, -283.9906568960454933, -329.2267048159183673 ) ) ;
#16819=CARTESIAN_POINT ( 'NONE',  ( 167.6033460894835514, 232.7025357865791761, -192.5994064317780499 ) ) ;
#16820=CARTESIAN_POINT ( 'NONE',  ( -40.96029181214492354, -138.9527141626594471, -363.1313459277565698 ) ) ;
#16821=CARTESIAN_POINT ( 'NONE',  ( 25.13358130842753013, -23.89985919551285320, -341.3865608528514031 ) ) ;
#16823=CARTESIAN_POINT ( 'NONE',  ( -7.451012908818240632, -275.8470437144422931, -337.1379743399647282 ) ) ;
#16824=CARTESIAN_POINT ( 'NONE',  ( -108.7906236507094206, -277.2561894567026002, -286.8264685628327015 ) ) ;
#16825=CARTESIAN_POINT ( 'NONE',  ( -63.54590728247134734, -273.3864835554318802, -197.9796022558082882 ) ) ;
#16826=CARTESIAN_POINT ( 'NONE',  ( 203.9605994126933695, 292.2036918473053220, -68.32866313698069405 ) ) ;
#16827=CARTESIAN_POINT ( 'NONE',  ( -38.55404822206283910, -275.7518882384251810, -346.8583629442123311 ) ) ;
#16828=CARTESIAN_POINT ( 'NONE',  ( -80.43875371432221755, -290.1461233899415788, -329.4209539967401383 ) ) ;
#16829=CARTESIAN_POINT ( 'NONE',  ( -35.48704261382476943, -298.8776464955855658, -193.5223475898178549 ) ) ;
#16830=CARTESIAN_POINT ( 'NONE',  ( 34.48912959104492160, -286.4413584485577076, -285.9627722571166828 ) ) ;
#16831=CARTESIAN_POINT ( 'NONE',  ( 99.04417061415693979, -300.2092272999767033, -193.4114905176868149 ) ) ;
#16832=CARTESIAN_POINT ( 'NONE',  ( -110.0505154012976163, -296.8119577760729726, -263.3017666189052193 ) ) ;
#16835=CARTESIAN_POINT ( 'NONE',  ( -53.79344272909299463, -279.1817131675209680, -344.1619658531067216 ) ) ;
#16837=CARTESIAN_POINT ( 'NONE',  ( -1.668243368071833821, -282.0998355195338831, -338.5295225861873405 ) ) ;
#16838=CARTESIAN_POINT ( 'NONE',  ( -108.7844176582288327, -279.4151824684268490, -286.8533776154830548 ) ) ;
#16839=CARTESIAN_POINT ( 'NONE',  ( -95.36076508472488911, -279.6421329664875657, -319.4501461133698967 ) ) ;
#16840=CARTESIAN_POINT ( 'NONE',  ( -94.05615359452258417, -295.7865274240317035, -223.4496692724162870 ) ) ;
#16842=CARTESIAN_POINT ( 'NONE',  ( -70.94355735715795674, -279.7625603924687425, -205.5402776106506622 ) ) ;
#16843=CARTESIAN_POINT ( 'NONE',  ( -93.06212646645815312, -274.0797348978318269, -217.4326247039715270 ) ) ;
#16844=CARTESIAN_POINT ( 'NONE',  ( -99.56392702124611560, -275.1197216753007524, -228.3950538420398004 ) ) ;
#16845=CARTESIAN_POINT ( 'NONE',  ( 39.03359027425954508, -274.1731683567476807, -274.0338826733132578 ) ) ;
#16848=CARTESIAN_POINT ( 'NONE',  ( -20.02404909225396779, -291.4774799949723274, -199.2263798403705266 ) ) ;
#16850=CARTESIAN_POINT ( 'NONE',  ( -114.2387934545425736, -283.9055874384102935, -269.9740466585116110 ) ) ;
#16851=CARTESIAN_POINT ( 'NONE',  ( 36.14312662533373555, -279.9123008192329962, -279.6067568330414019 ) ) ;
#16852=CARTESIAN_POINT ( 'NONE',  ( 27.36459976079593659, -280.6012912615097434, -305.4106496532297683 ) ) ;
#16853=CARTESIAN_POINT ( 'NONE',  ( -65.61799331073812880, -283.7594678311130565, -201.4457799542879286 ) ) ;
#16854=CARTESIAN_POINT ( 'NONE',  ( -84.11119433614436502, -291.6947761890994002, -329.0579476218634909 ) ) ;
#16855=CARTESIAN_POINT ( 'NONE',  ( 34.95558081160879027, -282.5911506183376218, -257.7027739279262732 ) ) ;
#16856=CARTESIAN_POINT ( 'NONE',  ( -106.2301241842228308, -270.9413509115434522, -240.5754438293160149 ) ) ;
#16857=CARTESIAN_POINT ( 'NONE',  ( -55.53116528385956485, -281.6823283391320842, -344.3583055693906658 ) ) ;
#16858=CARTESIAN_POINT ( 'NONE',  ( 36.11698851220483419, -295.7465373086176328, -285.4879721039424680 ) ) ;
#16859=CARTESIAN_POINT ( 'NONE',  ( -108.6474046387803440, -277.1300437811896700, -243.9515604728954656 ) ) ;
#16860=CARTESIAN_POINT ( 'NONE',  ( -109.1418353169747064, -279.0217701751894310, -284.1616016910651297 ) ) ;
#16861=CARTESIAN_POINT ( 'NONE',  ( -106.2557460714628661, -286.9457713853567498, -240.2161653820762695 ) ) ;
#16863=CARTESIAN_POINT ( 'NONE',  ( -40.59535378736537581, -293.9317136983653427, -194.8582630164650880 ) ) ;
#16864=CARTESIAN_POINT ( 'NONE',  ( 35.83930168603148303, -273.7635456023746201, -286.8371525849747741 ) ) ;
#16865=CARTESIAN_POINT ( 'NONE',  ( -37.51151711632554253, -288.2513631695539971, -347.2124989055708397 ) ) ;
#16866=CARTESIAN_POINT ( 'NONE',  ( -19.86314770634546534, -290.6803124781857832, -198.6079194367765695 ) ) ;
#16868=CARTESIAN_POINT ( 'NONE',  ( -56.74639997845254413, -275.9923087602757619, -341.2991004499526753 ) ) ;
#16869=CARTESIAN_POINT ( 'NONE',  ( -98.20951097852338307, -294.1090690068904792, -312.8578835477728717 ) ) ;
#16870=CARTESIAN_POINT ( 'NONE',  ( -87.05069338917586208, -291.0766277584838235, -324.5620117508524913 ) ) ;
#16873=CARTESIAN_POINT ( 'NONE',  ( 34.82432513934203655, -292.3492107278763683, -295.3175258151670732 ) ) ;
#16874=CARTESIAN_POINT ( 'NONE',  ( -4.253955750511765110, -288.0960080642899470, -204.3941445083287078 ) ) ;
#16875=CARTESIAN_POINT ( 'NONE',  ( 20.70030373011753255, -286.4615711264362972, -319.4029348769312264 ) ) ;
#16876=CARTESIAN_POINT ( 'NONE',  ( -46.81859243323795994, -287.3548901905036246, -197.3334738958409105 ) ) ;
#16878=CARTESIAN_POINT ( 'NONE',  ( 34.15162943915060367, -288.1505195896593250, -254.8271051424618179 ) ) ;
#16879=CARTESIAN_POINT ( 'NONE',  ( -27.92776968259137504, -296.9132276242093553, -345.1781358930899728 ) ) ;
#16881=CARTESIAN_POINT ( 'NONE',  ( 18.05369029194578445, -288.0292381278296716, -217.3756621137121385 ) ) ;
#16882=CARTESIAN_POINT ( 'NONE',  ( -98.49891727662877372, -276.0318235976262713, -314.7577717115177052 ) ) ;
#16884=CARTESIAN_POINT ( 'NONE',  ( -20.12670252300265261, -277.1702008765964251, -345.4450711649213304 ) ) ;
#16886=CARTESIAN_POINT ( 'NONE',  ( -38.16542169287795616, -279.7088143624405348, -193.3866691411668057 ) ) ;
#16887=CARTESIAN_POINT ( 'NONE',  ( -109.4305729840638719, -298.7827682100736411, -250.9458196565193475 ) ) ;
#16888=CARTESIAN_POINT ( 'NONE',  ( -38.63451889773383385, -284.0358156024701657, -195.3594330193917017 ) ) ;
#16890=CARTESIAN_POINT ( 'NONE',  ( -86.28100845742068259, -277.5039957914335673, -214.5416807046806582 ) ) ;
#16891=CARTESIAN_POINT ( 'NONE',  ( -94.75614194888153463, -281.8847434534070544, -318.6363861277664000 ) ) ;
#16893=CARTESIAN_POINT ( 'NONE',  ( 35.39582863089869846, -274.3245680970852050, -293.4253687317366825 ) ) ;
#16895=CARTESIAN_POINT ( 'NONE',  ( -110.9330423195532802, -298.0216338201580584, -274.2369540547595648 ) ) ;
#16896=CARTESIAN_POINT ( 'NONE',  ( 9.011003509519834864, -281.3529022378045283, -331.4587396578206722 ) ) ;
#16897=CARTESIAN_POINT ( 'NONE',  ( -108.7090245018078605, -297.7095169347002184, -253.9259891209473210 ) ) ;
#16898=CARTESIAN_POINT ( 'NONE',  ( -30.55593340486651499, -299.4506030025160044, -193.8527844494389853 ) ) ;
#16899=CARTESIAN_POINT ( 'NONE',  ( 7.347200606675306389, -274.3476551295489116, -212.6117488275851883 ) ) ;
#16900=CARTESIAN_POINT ( 'NONE',  ( -8.994538752723119757, -294.4228991626841321, -200.8692857695782834 ) ) ;
#16901=CARTESIAN_POINT ( 'NONE',  ( 35.84836915531595025, -287.4159530325503624, -246.2696239121606823 ) ) ;
#16902=CARTESIAN_POINT ( 'NONE',  ( -66.77848234817165007, -277.7493132929823787, -200.7709602571649725 ) ) ;
#16903=CARTESIAN_POINT ( 'NONE',  ( -111.9940479367977133, -290.6221652319840132, -251.4393380131373306 ) ) ;
#16905=CARTESIAN_POINT ( 'NONE',  ( -37.27981480475732212, -288.1101049069158648, -343.5963869393783057 ) ) ;
#16906=CARTESIAN_POINT ( 'NONE',  ( 36.10666853762655393, -291.7468634865115291, -285.5380014803782842 ) ) ;
#16909=CARTESIAN_POINT ( 'NONE',  ( -83.86340288714998792, -290.9005038762270487, -214.0253423701204269 ) ) ;
#16911=CARTESIAN_POINT ( 'NONE',  ( -114.0918971416658962, -285.5338572645170530, -267.1362844392434113 ) ) ;
#16912=CARTESIAN_POINT ( 'NONE',  ( 15.28560599361442485, -291.8322407444836131, -214.4026413756341185 ) ) ;
#16913=CARTESIAN_POINT ( 'NONE',  ( -21.80963834105200050, -284.1722620795108014, -345.2747571151184047 ) ) ;
#16914=CARTESIAN_POINT ( 'NONE',  ( 5.590377952295035868, -282.2854313356813805, -329.4020925357089027 ) ) ;
#16915=CARTESIAN_POINT ( 'NONE',  ( -73.28062652725911619, -297.5893465982373982, -202.2038613488620911 ) ) ;
#16916=CARTESIAN_POINT ( 'NONE',  ( 7.619485114162730000, -275.9958450415558673, -212.2256271169063098 ) ) ;
#16917=CARTESIAN_POINT ( 'NONE',  ( -52.68374753490112994, -289.8748662645199374, -197.2569162825540730 ) ) ;
#16918=CARTESIAN_POINT ( 'NONE',  ( -0.3328679173530076918, -273.3509390518309488, -206.9628769600639941 ) ) ;
#16919=ORIENTED_EDGE ( 'NONE', *, *, #31936, .T. ) ;
#16921=CARTESIAN_POINT ( 'NONE',  ( -27.67326489559168223, -288.0960660726323681, -196.5516635986635947 ) ) ;
#16922=CARTESIAN_POINT ( 'NONE',  ( -112.8969232000900007, -297.4629437503029976, -283.8100765555144562 ) ) ;
#16923=CARTESIAN_POINT ( 'NONE',  ( -110.1966776930315461, -285.1244803057439867, -276.3648594812455599 ) ) ;
#16924=CARTESIAN_POINT ( 'NONE',  ( -109.5196416438047891, -277.2780177737372469, -296.6541101900322133 ) ) ;
#16925=CARTESIAN_POINT ( 'NONE',  ( 38.71695036450618232, -294.3454622809013586, -281.6922464279305700 ) ) ;
#16926=CARTESIAN_POINT ( 'NONE',  ( 38.11510842493029827, -285.7784793148747440, -277.1857441102209236 ) ) ;
#16927=CARTESIAN_POINT ( 'NONE',  ( 22.27295568578142237, -294.5395298214356217, -319.0833229039461116 ) ) ;
#16928=CARTESIAN_POINT ( 'NONE',  ( -104.7242202130908453, -291.2643261286660277, -242.0926473140400788 ) ) ;
#16929=DIRECTION ( 'NONE',  ( 0.9951408606192334583, 0.000000000000000000, -0.09846150276129006507 ) ) ;
#16931=CARTESIAN_POINT ( 'NONE',  ( 138.9826652911064855, 178.1392901162842577, -238.3061235048771778 ) ) ;
#16932=CARTESIAN_POINT ( 'NONE',  ( -108.3900794218999692, -286.4299457453257673, -242.3814567359070509 ) ) ;
#16933=CARTESIAN_POINT ( 'NONE',  ( 13.84574458161073807, -278.1952119285919025, -206.2264541496106460 ) ) ;
#16935=CARTESIAN_POINT ( 'NONE',  ( -71.56532022638916146, -282.4358446507671374, -335.1914342064756624 ) ) ;
#16936=CARTESIAN_POINT ( 'NONE',  ( -100.4506040249524261, -277.6360247024985597, -314.4407112256638470 ) ) ;
#16937=CARTESIAN_POINT ( 'NONE',  ( 14.58947640107679078, -282.7847647473660686, -216.4077518846299881 ) ) ;
#16938=CARTESIAN_POINT ( 'NONE',  ( -28.98919269380465735, -125.6596419279838699, -362.8013170975748949 ) ) ;
#16939=CARTESIAN_POINT ( 'NONE',  ( -8.279932611388820973, -281.2538601208498221, -341.0855979981232053 ) ) ;
#16940=CARTESIAN_POINT ( 'NONE',  ( 21.65582614244480553, -284.9424047584124082, -224.6321479469126245 ) ) ;
#16941=CARTESIAN_POINT ( 'NONE',  ( -24.39437530483978733, -276.0760082679493053, -195.6574900559521382 ) ) ;
#16942=CARTESIAN_POINT ( 'NONE',  ( -34.29235569821962315, -295.5051301439532381, -343.3589942553924743 ) ) ;
#16943=CARTESIAN_POINT ( 'NONE',  ( 19.73933626591457369, -291.5862391993420601, -224.0486734630941328 ) ) ;
#16944=CARTESIAN_POINT ( 'NONE',  ( -113.1972525816878345, -279.0455311966885006, -282.9804661692281798 ) ) ;
#16945=CARTESIAN_POINT ( 'NONE',  ( -1.470229989576658847, -276.5627249245064263, -333.9969134662892429 ) ) ;
#16946=CARTESIAN_POINT ( 'NONE',  ( 23.39648751719547803, -273.8448675966208157, -223.5170397119977963 ) ) ;
#16947=CARTESIAN_POINT ( 'NONE',  ( 24.96937360118007021, -22.70870616268144815, -344.9910381550471925 ) ) ;
#16948=CARTESIAN_POINT ( 'NONE',  ( -66.11645737103935971, -275.4285525426614640, -339.6353506295643001 ) ) ;
#16949=CARTESIAN_POINT ( 'NONE',  ( -58.66931876783620226, -296.7478338671903657, -343.7902274546861463 ) ) ;
#16954=CARTESIAN_POINT ( 'NONE',  ( -109.2801883229806776, -285.4464827773321076, -284.4706888701941807 ) ) ;
#16955=CARTESIAN_POINT ( 'NONE',  ( -102.0433469577533856, -285.7845322712520328, -310.2067063202604800 ) ) ;
#16956=CARTESIAN_POINT ( 'NONE',  ( 16.97190299059360896, -286.2009674662938892, -221.4146730290349012 ) ) ;
#16957=CARTESIAN_POINT ( 'NONE',  ( -3.518778747445463928, -274.9977535096032852, -335.9541847371747849 ) ) ;
#16958=CARTESIAN_POINT ( 'NONE',  ( 34.52517894979501278, -283.6546429237428697, -289.0133525352189281 ) ) ;
#16959=CARTESIAN_POINT ( 'NONE',  ( -83.45555153473983978, -276.1771355168610853, -327.9091566341014641 ) ) ;
#16960=CARTESIAN_POINT ( 'NONE',  ( -45.93072475215929273, -278.2431532691024927, -343.2161796017575170 ) ) ;
#16963=CARTESIAN_POINT ( 'NONE',  ( 39.24993377288539875, -282.2778480708300890, -264.2064095004320734 ) ) ;
#16964=CARTESIAN_POINT ( 'NONE',  ( -11.53590649010932090, -280.8716521232119021, -197.8235441082313457 ) ) ;
#16968=CARTESIAN_POINT ( 'NONE',  ( -13.12136136878560677, -288.2239406534709474, -198.5719776515869341 ) ) ;
#16969=CARTESIAN_POINT ( 'NONE',  ( -55.32348060182023630, -297.0121430608490414, -199.3914370556261986 ) ) ;
#16971=CARTESIAN_POINT ( 'NONE',  ( -66.96849824421387609, -291.0224863172368828, -199.3993985831009752 ) ) ;
#16972=CARTESIAN_POINT ( 'NONE',  ( 32.94061699415235722, -285.7405323709311915, -248.1579772003571804 ) ) ;
#16973=CARTESIAN_POINT ( 'NONE',  ( -13.11084249534434676, -287.3057883155887566, -339.8466593202759327 ) ) ;
#16974=CARTESIAN_POINT ( 'NONE',  ( -25.22137191851076921, -290.4484896307543522, -197.2947342759682954 ) ) ;
#16975=CARTESIAN_POINT ( 'NONE',  ( -73.76594619740265557, -286.7621236417540445, -206.6252358071488970 ) ) ;
#16976=CARTESIAN_POINT ( 'NONE',  ( -70.70467126983730566, -275.4920321204199922, -337.5318914601073175 ) ) ;
#16977=CARTESIAN_POINT ( 'NONE',  ( 34.31315527711925739, -286.2846074382899815, -296.4379081585745439 ) ) ;
#16978=CARTESIAN_POINT ( 'NONE',  ( 32.97016659585824527, -289.2135120769601144, -244.2605041038906108 ) ) ;
#16979=CARTESIAN_POINT ( 'NONE',  ( -100.7683000735515861, -288.0092793921699013, -310.7942131821229168 ) ) ;
#16980=CARTESIAN_POINT ( 'NONE',  ( 34.17276622843636602, -282.7009356366545489, -286.1436890870045318 ) ) ;
#16981=CARTESIAN_POINT ( 'NONE',  ( -111.3242141045046907, -292.3811216812559906, -283.7233813739512129 ) ) ;
#16982=CARTESIAN_POINT ( 'NONE',  ( 82.12627345295348391, -301.3282310295588218, -194.4389801081340750 ) ) ;
#16984=CARTESIAN_POINT ( 'NONE',  ( -108.5030666233512591, -298.7990811821818511, -244.9569034656359747 ) ) ;
#16985=CARTESIAN_POINT ( 'NONE',  ( -30.23654905568832874, -279.3413577191250852, -197.4950036532778768 ) ) ;
#16986=CARTESIAN_POINT ( 'NONE',  ( 37.42051237654314377, -279.6366088439660871, -276.9515588317134416 ) ) ;
#16987=CARTESIAN_POINT ( 'NONE',  ( 39.07534425039197856, -292.8561752934695619, -278.8871293087453864 ) ) ;
#16988=CARTESIAN_POINT ( 'NONE',  ( -55.47068109827161919, -296.2149755502882158, -198.7695741559975886 ) ) ;
#16989=CARTESIAN_POINT ( 'NONE',  ( 8.447282414967718367, -274.4999384803279554, -329.1182074055128055 ) ) ;
#16990=CARTESIAN_POINT ( 'NONE',  ( -42.40710803614312852, -296.4325490641732017, -343.6794998601117186 ) ) ;
#16992=CARTESIAN_POINT ( 'NONE',  ( -106.3035797775020939, -271.5520077986109868, -237.4541970312146475 ) ) ;
#16993=CARTESIAN_POINT ( 'NONE',  ( -53.10126226642907454, -293.4912341868555359, -344.7493952095852023 ) ) ;
#16994=CARTESIAN_POINT ( 'NONE',  ( 4.826547729575792367, -294.0591414711578864, -209.9893452760917683 ) ) ;
#16996=CARTESIAN_POINT ( 'NONE',  ( -5.981666331252039726, -293.2780588215939588, -204.2477605534664633 ) ) ;
#16997=FACE_OUTER_BOUND ( 'NONE', #53513, .T. ) ;
#16998=CARTESIAN_POINT ( 'NONE',  ( -112.6958619816320777, -282.5773222533448461, -269.9647708052559665 ) ) ;
#16999=CARTESIAN_POINT ( 'NONE',  ( -31.60235537226621716, -294.9778227182930550, -343.1852644781941422 ) ) ;
#17000=CARTESIAN_POINT ( 'NONE',  ( -41.56913770093522942, -283.1038741220709767, -347.2973100054052793 ) ) ;
#17001=CARTESIAN_POINT ( 'NONE',  ( 37.74880882459412135, -283.3592998368132498, -261.4942062133706600 ) ) ;
#17002=CARTESIAN_POINT ( 'NONE',  ( -3.494824020551794419, -286.1534599689020411, -201.2080857129227809 ) ) ;
#17003=CARTESIAN_POINT ( 'NONE',  ( -109.5134422913925221, -288.8069350189473425, -250.5806209750258233 ) ) ;
#17004=CARTESIAN_POINT ( 'NONE',  ( 6.510594546088531942, -280.9483687434054673, -332.8731700484629528 ) ) ;
#17005=CARTESIAN_POINT ( 'NONE',  ( 20.74062453112327731, -285.6070153726224703, -225.3312718612742742 ) ) ;
#17006=CARTESIAN_POINT ( 'NONE',  ( 38.67072726555026208, -286.3446736192034336, -260.1825428703251646 ) ) ;
#17008=CARTESIAN_POINT ( 'NONE',  ( -73.67874856097451186, -297.1432550405769462, -334.5955271957656123 ) ) ;
#17009=CARTESIAN_POINT ( 'NONE',  ( -94.75596750805311785, -279.2898065592671628, -320.7814332830569128 ) ) ;
#17010=CARTESIAN_POINT ( 'NONE',  ( 35.85614590610301633, -291.8017124174068613, -288.3170494176977741 ) ) ;
#17011=CARTESIAN_POINT ( 'NONE',  ( -98.00880881844318537, -278.7842456769117234, -229.6315892427783751 ) ) ;
#17012=CARTESIAN_POINT ( 'NONE',  ( 24.81319831579656210, -293.1153996583991557, -224.9103907721864459 ) ) ;
#17013=CARTESIAN_POINT ( 'NONE',  ( -57.35062240519914667, -283.8758860046265227, -197.4442149746326436 ) ) ;
#17014=CARTESIAN_POINT ( 'NONE',  ( -20.54848316024892085, -278.8368119783942802, -343.5101689620825596 ) ) ;
#17015=CARTESIAN_POINT ( 'NONE',  ( -86.65723617984265559, -294.8168589714524046, -324.5033967625814171 ) ) ;
#17017=CARTESIAN_POINT ( 'NONE',  ( -62.15860923440826014, -295.7292613177100975, -199.5859693065293925 ) ) ;
#17021=CARTESIAN_POINT ( 'NONE',  ( 16.42706245153227584, -282.8001759990223150, -218.5111828052056069 ) ) ;
#17022=CARTESIAN_POINT ( 'NONE',  ( -110.3034514814425933, -296.0094886284684321, -274.1783527068847661 ) ) ;
#17024=CARTESIAN_POINT ( 'NONE',  ( 35.77081079830085031, -273.2666405000204009, -287.0812184334320705 ) ) ;
#17025=CARTESIAN_POINT ( 'NONE',  ( 7.149834651440080791, -273.8380913146555145, -207.6486904937819702 ) ) ;
#17029=CARTESIAN_POINT ( 'NONE',  ( 37.53736984938573329, -288.6689337078706217, -254.5998794257499185 ) ) ;
#17030=CARTESIAN_POINT ( 'NONE',  ( -21.13140423249311795, -288.6716417095884708, -341.5385463672683386 ) ) ;
#17032=CARTESIAN_POINT ( 'NONE',  ( -16.74632019806061933, -281.8432034523698348, -199.6042237854304062 ) ) ;
#17033=CARTESIAN_POINT ( 'NONE',  ( 9.714448960572047653, -300.4092151778905304, -196.3334390736784485 ) ) ;
#17034=CARTESIAN_POINT ( 'NONE',  ( -34.28149324702157941, -278.8863664845567314, -197.0152557882587985 ) ) ;
#17036=CARTESIAN_POINT ( 'NONE',  ( -40.43515626221180526, -297.6811161879879819, -193.3923310999386445 ) ) ;
#17037=CARTESIAN_POINT ( 'NONE',  ( -70.89118457865664880, -293.5261031612056399, -203.9100360180572409 ) ) ;
#17039=CARTESIAN_POINT ( 'NONE',  ( -102.9332448087500751, -290.7668413008985908, -302.6355960454165483 ) ) ;
#17041=CARTESIAN_POINT ( 'NONE',  ( -34.97487675231187154, -290.2211375274265492, -194.6203530960704882 ) ) ;
#17042=CARTESIAN_POINT ( 'NONE',  ( -94.46520784620715006, -296.8610407036135257, -224.8749403803518874 ) ) ;
#17044=CARTESIAN_POINT ( 'NONE',  ( -94.20765612706266268, -292.7686938366508684, -219.4791879710477929 ) ) ;
#17045=CARTESIAN_POINT ( 'NONE',  ( -99.86837403722181250, -298.4090924074129703, -320.2651865833026363 ) ) ;
#17046=CARTESIAN_POINT ( 'NONE',  ( 32.68129103810331060, -289.2069678638544588, -243.8178324011119855 ) ) ;
#17047=CARTESIAN_POINT ( 'NONE',  ( 6.449504501896194952, -274.4559377987663993, -331.1075355486583476 ) ) ;
#17048=CARTESIAN_POINT ( 'NONE',  ( 36.79023414869326558, -277.5598317763680143, -277.1265090728467158 ) ) ;
#17049=CARTESIAN_POINT ( 'NONE',  ( -19.70779079199753525, -290.3603383001662337, -197.9865895230953470 ) ) ;
#17050=CARTESIAN_POINT ( 'NONE',  ( -1.737187634855947405, -282.3792463229756322, -203.4834373066694297 ) ) ;
#17053=CARTESIAN_POINT ( 'NONE',  ( -1.208828318248188038, -281.9076789745990368, -333.9088027796296956 ) ) ;
#17054=CARTESIAN_POINT ( 'NONE',  ( -104.5294228811511914, -280.1126735611623531, -233.3840653657056805 ) ) ;
#17055=CARTESIAN_POINT ( 'NONE',  ( 30.71729914961442631, -280.8026177128979839, -305.5176441876676563 ) ) ;
#17056=CARTESIAN_POINT ( 'NONE',  ( -20.16704954168087482, -277.7780738584860956, -345.2344634095481410 ) ) ;
#17058=CARTESIAN_POINT ( 'NONE',  ( 22.20503976414471481, -276.4270353467877044, -222.6235991421189908 ) ) ;
#17059=CARTESIAN_POINT ( 'NONE',  ( -21.33282851196159058, -279.3376638359844719, -340.3538533559490702 ) ) ;
#17061=CARTESIAN_POINT ( 'NONE',  ( -112.3757206867542209, -298.5734697461911651, -268.7137049685347847 ) ) ;
#17062=CARTESIAN_POINT ( 'NONE',  ( -100.5635952833257676, -291.1231957957028271, -307.5719586288238929 ) ) ;
#17063=CARTESIAN_POINT ( 'NONE',  ( -62.40794291757152479, -291.1338337932824629, -342.1499922993866676 ) ) ;
#17064=CARTESIAN_POINT ( 'NONE',  ( -37.54191246908424517, -291.3982018185155880, -197.2469975106114077 ) ) ;
#17065=CARTESIAN_POINT ( 'NONE',  ( -9.591380266982669767, -288.2067576737762806, -342.1207629847342560 ) ) ;
#17067=CARTESIAN_POINT ( 'NONE',  ( -109.9768138420115662, -283.1233705359891815, -257.2294789445528522 ) ) ;
#17068=CARTESIAN_POINT ( 'NONE',  ( -98.35075614819106704, -291.8328144825426875, -312.6771825152179076 ) ) ;
#17069=CARTESIAN_POINT ( 'NONE',  ( -110.2958998249210509, -283.1680735061545988, -259.9499461383621224 ) ) ;
#17070=CARTESIAN_POINT ( 'NONE',  ( -27.50886567974005459, -281.4947197331291022, -197.4771800675971463 ) ) ;
#17071=CARTESIAN_POINT ( 'NONE',  ( 39.36982669833987103, -288.5440512768979033, -274.3985717569670442 ) ) ;
#17072=CARTESIAN_POINT ( 'NONE',  ( -85.52946810435238945, -279.8563801938807956, -215.4436575628681965 ) ) ;
#17073=CARTESIAN_POINT ( 'NONE',  ( -79.36370624807180718, -290.2937126527990017, -206.2496138276864315 ) ) ;
#17074=CARTESIAN_POINT ( 'NONE',  ( 39.44349999278087893, -288.4056541474216147, -274.4042232703071136 ) ) ;
#17075=CARTESIAN_POINT ( 'NONE',  ( 14.20099994950011357, -287.2454115821495293, -213.1680483020372776 ) ) ;
#17076=CARTESIAN_POINT ( 'NONE',  ( -93.42070761499181231, -284.0556817035841277, -317.0959542807008802 ) ) ;
#17077=ORIENTED_EDGE ( 'NONE', *, *, #25991, .F. ) ;
#17079=CARTESIAN_POINT ( 'NONE',  ( -35.02234885980617207, -293.9413678095104956, -194.6188838303984028 ) ) ;
#17081=CARTESIAN_POINT ( 'NONE',  ( 24.47785268041048568, -292.8393481070178836, -315.4569098001047678 ) ) ;
#17082=CARTESIAN_POINT ( 'NONE',  ( -21.61413719671539369, -275.9044262284627393, -341.9398599046951404 ) ) ;
#17083=CARTESIAN_POINT ( 'NONE',  ( -113.0373125896367412, -296.0703745083641252, -256.8153791377112611 ) ) ;
#17084=CARTESIAN_POINT ( 'NONE',  ( 22.37783350028307794, -291.4334531066760974, -227.1622849017408043 ) ) ;
#17085=CARTESIAN_POINT ( 'NONE',  ( -65.94389949280636642, -295.9125459065321593, -202.0977441553750111 ) ) ;
#17087=CARTESIAN_POINT ( 'NONE',  ( -14.73861911021209536, -293.5567719355829013, -200.5311012799999446 ) ) ;
#17088=CARTESIAN_POINT ( 'NONE',  ( 16.95792029340102047, -293.9283570217650663, -221.0345013277714372 ) ) ;
#17091=CARTESIAN_POINT ( 'NONE',  ( -73.74143771664761005, -293.5336571068012859, -336.1848155651765637 ) ) ;
#17092=CARTESIAN_POINT ( 'NONE',  ( -108.1383874600115860, -298.8746320690293601, -245.4521829112844387 ) ) ;
#17093=CARTESIAN_POINT ( 'NONE',  ( 5.993473317834490999, -289.3895814077063164, -329.4622047780503067 ) ) ;
#17096=CARTESIAN_POINT ( 'NONE',  ( -69.57408567824386125, -279.4541102137527560, -338.4889746555440979 ) ) ;
#17097=CARTESIAN_POINT ( 'NONE',  ( -64.96627987024398010, -276.1999092687393045, -341.8656412701643603 ) ) ;
#17098=CARTESIAN_POINT ( 'NONE',  ( -101.1193559776045845, -272.4685757678341247, -227.3044516608795220 ) ) ;
#17099=CARTESIAN_POINT ( 'NONE',  ( 33.35169860706576372, -279.3265370003301769, -246.8798789812441328 ) ) ;
#17100=CARTESIAN_POINT ( 'NONE',  ( -20.32479232698709737, -275.2371024213733222, -344.6908681440314695 ) ) ;
#17101=AXIS2_PLACEMENT_3D ( 'NONE', #80411, #73786, #58660 ) ;
#17102=CARTESIAN_POINT ( 'NONE',  ( -109.3713837463181164, -295.0449333588217087, -285.0172878133939776 ) ) ;
#17104=CARTESIAN_POINT ( 'NONE',  ( -91.20324744867943423, -273.9120753011823695, -220.9176282906345818 ) ) ;
#17106=CARTESIAN_POINT ( 'NONE',  ( -107.9241650482618553, -288.9150467175742847, -243.8208380544978411 ) ) ;
#17107=CARTESIAN_POINT ( 'NONE',  ( 34.62601386784767499, -275.2231172221764268, -258.0537830887010387 ) ) ;
#17109=CARTESIAN_POINT ( 'NONE',  ( 16.68595630013767206, -288.3094014086133825, -325.2988411975274516 ) ) ;
#17110=CARTESIAN_POINT ( 'NONE',  ( -37.62728611644039489, -300.0284796732971699, -195.0064548997399356 ) ) ;
#17111=CARTESIAN_POINT ( 'NONE',  ( -81.25057586038475677, -293.6504158035310184, -330.9584698689731681 ) ) ;
#17112=CARTESIAN_POINT ( 'NONE',  ( -44.41455641505240948, -282.3365025426542161, -346.9266734630156179 ) ) ;
#17114=CARTESIAN_POINT ( 'NONE',  ( 31.98991793651351401, -279.1772270529588127, -241.6243364124823358 ) ) ;
#17117=CARTESIAN_POINT ( 'NONE',  ( -100.0428952900193735, -289.8697157148333190, -232.2076039955548481 ) ) ;
#17118=CARTESIAN_POINT ( 'NONE',  ( -56.66282946885505112, -281.4434672721770880, -342.0378885477648510 ) ) ;
#17120=CARTESIAN_POINT ( 'NONE',  ( -110.9052975537900636, -288.3635819187505831, -285.0350590254873282 ) ) ;
#17121=CARTESIAN_POINT ( 'NONE',  ( 22.02837887884630064, -276.4663330344525320, -226.7044864991603674 ) ) ;
#17122=CARTESIAN_POINT ( 'NONE',  ( -1.804651291749928221, -283.7969840363227263, -338.2222031463684857 ) ) ;
#17123=CARTESIAN_POINT ( 'NONE',  ( -69.49632849633245257, -271.7122004015988637, -201.9701224755656881 ) ) ;
#17124=CARTESIAN_POINT ( 'NONE',  ( -82.79472189085720402, -283.6934346386124730, -327.5488571289008632 ) ) ;
#17125=CARTESIAN_POINT ( 'NONE',  ( 33.42163236142050664, -276.7103670143191607, -249.9820284977034532 ) ) ;
#17126=CARTESIAN_POINT ( 'NONE',  ( 32.67389097122043040, -276.6359001961558874, -291.6276374757095482 ) ) ;
#17127=CARTESIAN_POINT ( 'NONE',  ( 23.50016623585100106, -284.1495149351130181, -314.2380068539533795 ) ) ;
#17128=ORIENTED_EDGE ( 'NONE', *, *, #13516, .F. ) ;
#17130=CARTESIAN_POINT ( 'NONE',  ( 6.612260534475175255, -294.3063269520496306, -333.6483068051148848 ) ) ;
#17131=CARTESIAN_POINT ( 'NONE',  ( 35.30539193004074150, -289.3100312676060071, -253.1523306551676171 ) ) ;
#17133=CARTESIAN_POINT ( 'NONE',  ( -37.30987171927208834, -289.5523547857346784, -190.3611179825600175 ) ) ;
#17134=CARTESIAN_POINT ( 'NONE',  ( -112.4934941197131479, -277.2797112481852082, -285.7133348417480079 ) ) ;
#17136=CARTESIAN_POINT ( 'NONE',  ( -22.33122652777116812, -290.6410133030788074, -195.6004191284564797 ) ) ;
#17137=CARTESIAN_POINT ( 'NONE',  ( -110.7851798487517812, -285.9930491389008580, -276.4243710502900626 ) ) ;
#17138=CARTESIAN_POINT ( 'NONE',  ( -107.2135138095480897, -279.9901929397520348, -294.9275518852743971 ) ) ;
#17139=CARTESIAN_POINT ( 'NONE',  ( -108.4865581322787449, -286.3351113479791366, -242.3421374403021957 ) ) ;
#17140=CARTESIAN_POINT ( 'NONE',  ( -33.36539822217105922, -285.0022726118937726, -345.2685585424827082 ) ) ;
#17141=CARTESIAN_POINT ( 'NONE',  ( 30.54406808840042942, -276.1897650093678749, -306.8126993175403072 ) ) ;
#17142=CARTESIAN_POINT ( 'NONE',  ( -78.39603293036846310, -295.5172546557896567, -207.9581134579399304 ) ) ;
#17143=CARTESIAN_POINT ( 'NONE',  ( -82.23713664484530739, -279.2914289285507721, -207.8039458561275126 ) ) ;
#17144=CARTESIAN_POINT ( 'NONE',  ( -78.32478079314712716, -299.4166727202165248, -208.1565753724476338 ) ) ;
#17147=CARTESIAN_POINT ( 'NONE',  ( -113.3275340877688251, -270.8281558274566692, -267.5090283341868940 ) ) ;
#17150=CARTESIAN_POINT ( 'NONE',  ( -27.01901063854439045, -276.4250050130776799, -342.6897466384641575 ) ) ;
#17152=CARTESIAN_POINT ( 'NONE',  ( 15.74077815564904270, -275.9889201771181320, -215.1319661049836611 ) ) ;
#17153=CARTESIAN_POINT ( 'NONE',  ( 26.09296876122256492, -280.0379483352124907, -227.0380001738530495 ) ) ;
#17154=CARTESIAN_POINT ( 'NONE',  ( -0.4673932990832067036, -290.3154106884458088, -334.5937867421626493 ) ) ;
#17155=CARTESIAN_POINT ( 'NONE',  ( -81.45496320822191194, -297.1599595502635793, -332.6890176643797759 ) ) ;
#17156=CARTESIAN_POINT ( 'NONE',  ( -113.9685938274647015, -297.7306620818980605, -272.4742320110182163 ) ) ;
#17157=CARTESIAN_POINT ( 'NONE',  ( 12.12404266986732360, -294.7417573551070404, -214.1389104939089520 ) ) ;
#17158=CARTESIAN_POINT ( 'NONE',  ( 33.72551608239047027, -279.2465434817816572, -246.7566508464977915 ) ) ;
#17160=CARTESIAN_POINT ( 'NONE',  ( 8.000459377986219422, -282.5970605639263340, -211.2586148898205067 ) ) ;
#17161=CARTESIAN_POINT ( 'NONE',  ( -92.90373748404503829, -295.3267512501931265, -220.8214954148626816 ) ) ;
#17162=CARTESIAN_POINT ( 'NONE',  ( -110.7155831740642782, -285.8919349505402465, -290.9211204937889761 ) ) ;
#17163=CARTESIAN_POINT ( 'NONE',  ( 31.26874127271732462, -286.1276320056451823, -244.3946287249266049 ) ) ;
#17164=CARTESIAN_POINT ( 'NONE',  ( 191.3253626393375839, 269.8902699472227482, -139.2695367922076741 ) ) ;
#17166=CARTESIAN_POINT ( 'NONE',  ( 32.32019631698473461, -286.5310452160484260, -301.7589917162479765 ) ) ;
#17167=CARTESIAN_POINT ( 'NONE',  ( -8.242622313618772623, -286.1107520854085351, -203.3885030031145789 ) ) ;
#17169=CARTESIAN_POINT ( 'NONE',  ( -96.92351360873561816, -284.9813569728678431, -318.6673595311115150 ) ) ;
#17171=CARTESIAN_POINT ( 'NONE',  ( 26.78735444693427326, -276.3632556239281257, -305.3889150724034494 ) ) ;
#17172=CARTESIAN_POINT ( 'NONE',  ( -61.57780627145452712, -290.6649599033058848, -197.5445987055869637 ) ) ;
#17173=CARTESIAN_POINT ( 'NONE',  ( 38.32675761814055448, -282.3760011066274842, -284.1309160592298895 ) ) ;
#17175=CARTESIAN_POINT ( 'NONE',  ( -98.88029927190306978, -280.6771413161891360, -225.2202311764013416 ) ) ;
#17176=CARTESIAN_POINT ( 'NONE',  ( 37.30971162058846602, -281.6503181819015822, -251.5751919858336692 ) ) ;
#17177=CARTESIAN_POINT ( 'NONE',  ( 21.27581636871891391, -273.6952119285918457, -317.1477375740089997 ) ) ;
#17178=CARTESIAN_POINT ( 'NONE',  ( 190.4687118359351246, 271.0561473682616906, -139.6585402428168834 ) ) ;
#17180=CARTESIAN_POINT ( 'NONE',  ( 20.61730575103503682, -278.2062920943478730, -317.7182191956979977 ) ) ;
#17181=CARTESIAN_POINT ( 'NONE',  ( -48.94245970541811630, -154.4817453298226724, -364.6946769374113160 ) ) ;
#17183=CARTESIAN_POINT ( 'NONE',  ( 8.164578208348435950, -278.6976418584205248, -211.1262394462077907 ) ) ;
#17184=CARTESIAN_POINT ( 'NONE',  ( -44.57092174185743261, -297.3069882586909216, -197.5670679431429448 ) ) ;
#17185=CARTESIAN_POINT ( 'NONE',  ( 19.47999444693757454, -293.7663245176897249, -322.3118442344506320 ) ) ;
#17187=EDGE_CURVE ( 'NONE', #39736, #93199, #5012, .T. ) ;
#17188=CARTESIAN_POINT ( 'NONE',  ( -96.87575768589123015, -295.7738000571590078, -222.4622423559597735 ) ) ;
#17189=CARTESIAN_POINT ( 'NONE',  ( -109.7273595455288699, -288.7635493391237560, -284.8048825290147192 ) ) ;
#17190=CARTESIAN_POINT ( 'NONE',  ( -87.30410741372166683, -297.6180757882747798, -325.2667036394243496 ) ) ;
#17191=CARTESIAN_POINT ( 'NONE',  ( -14.42804321940216816, -287.6705714765064954, -200.4778971785131603 ) ) ;
#17193=CARTESIAN_POINT ( 'NONE',  ( 26.32332190230625457, -295.0602113281535708, -313.2515036511420021 ) ) ;
#17194=CARTESIAN_POINT ( 'NONE',  ( -110.1565851648223600, -284.9654399085665659, -276.3595309915473877 ) ) ;
#17195=CARTESIAN_POINT ( 'NONE',  ( -34.05265601491269933, -296.8874001566717880, -193.7588436825993483 ) ) ;
#17196=CARTESIAN_POINT ( 'NONE',  ( -56.15915852686629961, -292.6186911709002061, -195.8075443401529583 ) ) ;
#17197=CARTESIAN_POINT ( 'NONE',  ( -37.80095905698929926, -292.5388885756004242, -193.4240268963659730 ) ) ;
#17198=CARTESIAN_POINT ( 'NONE',  ( -106.0318524081430525, -290.3897157999033425, -295.0727141316814368 ) ) ;
#17201=CARTESIAN_POINT ( 'NONE',  ( -96.39867958376001411, -299.0589563173783176, -222.8997793745646163 ) ) ;
#17202=CARTESIAN_POINT ( 'NONE',  ( -34.10453689298036295, -272.8869472936946750, -193.8266192675493471 ) ) ;
#17203=CARTESIAN_POINT ( 'NONE',  ( -21.34846707110369124, -281.9008480602296913, -341.8809463694336728 ) ) ;
#17205=CARTESIAN_POINT ( 'NONE',  ( 1.010911956846083593, -276.0626131661437057, -337.1194019614455897 ) ) ;
#17206=CARTESIAN_POINT ( 'NONE',  ( 52.75270939764214262, -297.6798444388553548, -196.6916333512348842 ) ) ;
#17207=CARTESIAN_POINT ( 'NONE',  ( -103.2634827769061303, -280.8703711655966799, -236.1143822342512522 ) ) ;
#17208=CARTESIAN_POINT ( 'NONE',  ( -3.322169788990462891, -274.7375080479140479, -336.3424565439934781 ) ) ;
#17209=CARTESIAN_POINT ( 'NONE',  ( -108.8674280392905018, -297.9732979522711958, -253.8929440394740880 ) ) ;
#17210=CARTESIAN_POINT ( 'NONE',  ( -31.33231338057652948, -275.0711317793014814, -197.3601017455594899 ) ) ;
#17211=CARTESIAN_POINT ( 'NONE',  ( -97.61385962893201906, -298.7814247593959180, -223.7170187164452955 ) ) ;
#17212=CARTESIAN_POINT ( 'NONE',  ( 25.57152109108438864, -273.0149701683577064, -228.8842159966131646 ) ) ;
#17213=CARTESIAN_POINT ( 'NONE',  ( 18.54916894175702780, -293.5350613617497970, -223.2431445211967116 ) ) ;
#17214=CARTESIAN_POINT ( 'NONE',  ( -9.487757388262888725, -290.9980194240793594, -202.1927760936629284 ) ) ;
#17216=CARTESIAN_POINT ( 'NONE',  ( 5.841927170023497595, -276.9759802325876308, -334.0376539787597494 ) ) ;
#17217=CARTESIAN_POINT ( 'NONE',  ( -109.8860041760852653, -272.8262653978995900, -262.2171659512544011 ) ) ;
#17218=CARTESIAN_POINT ( 'NONE',  ( -10.88836768577169956, -281.3993021718861200, -342.2054139834787634 ) ) ;
#17219=CARTESIAN_POINT ( 'NONE',  ( -16.97846349042401570, -296.7901157069783835, -342.7708777124528297 ) ) ;
#17221=CARTESIAN_POINT ( 'NONE',  ( -92.68797249353914935, -283.0689085516376053, -318.2277759773480739 ) ) ;
#17222=CARTESIAN_POINT ( 'NONE',  ( -108.4975852124747746, -282.2393248533763881, -294.5864857530026484 ) ) ;
#17223=CARTESIAN_POINT ( 'NONE',  ( 25.79059335920872087, -273.6097927646864036, -232.4511574014176745 ) ) ;
#17224=CARTESIAN_POINT ( 'NONE',  ( -26.53897922994619307, -282.1896313915731866, -196.0916231665542000 ) ) ;
#17227=CARTESIAN_POINT ( 'NONE',  ( -91.58513040497733471, -271.6949018009564156, -216.8439180699880637 ) ) ;
#17229=CARTESIAN_POINT ( 'NONE',  ( -107.8944406815436849, -280.8897397468701342, -244.2812028689015165 ) ) ;
#17232=CARTESIAN_POINT ( 'NONE',  ( -86.82570441288859797, -287.2906765238827234, -213.1897511470764925 ) ) ;
#17234=CARTESIAN_POINT ( 'NONE',  ( -61.69377627843048373, -289.7356952099895580, -199.3705103345685927 ) ) ;
#17236=CARTESIAN_POINT ( 'NONE',  ( -108.3576466698271616, -295.1029814045311923, -288.9544704216328341 ) ) ;
#17237=CARTESIAN_POINT ( 'NONE',  ( -99.15205147371868577, -288.1302655786844298, -311.4980874790892926 ) ) ;
#17238=CARTESIAN_POINT ( 'NONE',  ( 188.7508426036948208, 279.9709457756753181, -124.8390596414617590 ) ) ;
#17239=CARTESIAN_POINT ( 'NONE',  ( -109.9110596246630251, -294.3080251905764726, -289.3510415761517152 ) ) ;
#17240=CARTESIAN_POINT ( 'NONE',  ( 29.53334351106362732, -285.5505582073838582, -233.5031484245756133 ) ) ;
#17241=CARTESIAN_POINT ( 'NONE',  ( 25.81042619173718577, -282.6311508200469120, -232.0750983725606602 ) ) ;
#17242=CARTESIAN_POINT ( 'NONE',  ( -106.0983797336095904, -282.3721391996784860, -302.7106623519830464 ) ) ;
#17243=CARTESIAN_POINT ( 'NONE',  ( -109.6229496821357969, -290.4161680802360479, -280.6694549657781863 ) ) ;
#17246=CARTESIAN_POINT ( 'NONE',  ( 29.50034846094592211, -282.5640185884734592, -239.4573254970343044 ) ) ;
#17247=CARTESIAN_POINT ( 'NONE',  ( -1.163283040704384375, -283.3616900024941287, -333.9513991910898199 ) ) ;
#17249=CARTESIAN_POINT ( 'NONE',  ( 37.71154575191060587, -289.6181687691748721, -277.1003378065689162 ) ) ;
#17250=CARTESIAN_POINT ( 'NONE',  ( -113.5240099626964394, -273.0281573994048472, -258.9520543865493778 ) ) ;
#17253=CARTESIAN_POINT ( 'NONE',  ( 37.59186835044970110, -275.7744047437907398, -288.1368362308884912 ) ) ;
#17254=CARTESIAN_POINT ( 'NONE',  ( -6.615725236069108561, -294.4374966344255995, -202.3334671863436824 ) ) ;
#17256=CARTESIAN_POINT ( 'NONE',  ( 21.27581636871892101, -289.4090924074130839, -223.5744983911110353 ) ) ;
#17257=CARTESIAN_POINT ( 'NONE',  ( 34.30721672438074421, -273.8446070346852821, -293.0868993893792549 ) ) ;
#17259=CARTESIAN_POINT ( 'NONE',  ( -48.82905715762767329, -296.3081915587064259, -194.9788592001873440 ) ) ;
#17260=CARTESIAN_POINT ( 'NONE',  ( -44.39675081950817059, -293.5617031899628273, -196.8477340852852535 ) ) ;
#17261=CARTESIAN_POINT ( 'NONE',  ( -19.23836903881461069, -273.6397564751534901, -199.4837471376149836 ) ) ;
#17262=CARTESIAN_POINT ( 'NONE',  ( -82.16596912329586644, -292.9485735068852819, -211.8030051529857474 ) ) ;
#17264=CARTESIAN_POINT ( 'NONE',  ( -94.48199854818197707, -292.1389076526286317, -224.5329478163124293 ) ) ;
#17265=CARTESIAN_POINT ( 'NONE',  ( -111.1038514978274065, -286.2330297360794020, -276.4536574495593300 ) ) ;
#17266=CARTESIAN_POINT ( 'NONE',  ( -113.7798749128485696, -292.0022879758289491, -268.3881773732959459 ) ) ;
#17267=CARTESIAN_POINT ( 'NONE',  ( -36.40136205443786821, -293.3788782935071140, -193.8470972502124994 ) ) ;
#17268=CARTESIAN_POINT ( 'NONE',  ( 22.93179133425186578, -293.9595900672553057, -311.6333210305399462 ) ) ;
#17269=CARTESIAN_POINT ( 'NONE',  ( 36.25146153568864094, -289.7388097368263402, -284.8860849424076491 ) ) ;
#17270=CARTESIAN_POINT ( 'NONE',  ( 36.47928983743612008, -281.9956219583908137, -292.4411704231692966 ) ) ;
#17271=CARTESIAN_POINT ( 'NONE',  ( 51.50024267128915056, -297.2358502085104988, -194.8298982140941575 ) ) ;
#17272=CARTESIAN_POINT ( 'NONE',  ( -111.1085870955612336, -284.1078938614560911, -292.4850959667163579 ) ) ;
#17273=CARTESIAN_POINT ( 'NONE',  ( 35.78079552368199501, -277.7255356919781661, -285.3593657375697603 ) ) ;
#17275=CARTESIAN_POINT ( 'NONE',  ( -96.24955757627314767, -282.7362816921143462, -314.1446175757996571 ) ) ;
#17276=CARTESIAN_POINT ( 'NONE',  ( 28.39128983025559805, -285.0705969506945507, -234.1399340539306024 ) ) ;
#17277=CARTESIAN_POINT ( 'NONE',  ( -14.97728027383291405, -274.9052119461082953, -342.8048412693465252 ) ) ;
#17279=CARTESIAN_POINT ( 'NONE',  ( -45.65269004266314568, -282.6678403796090606, -342.9994538287614319 ) ) ;
#17280=CARTESIAN_POINT ( 'NONE',  ( -73.59135694896299640, -280.7871346000828794, -202.8631258503381503 ) ) ;
#17281=CARTESIAN_POINT ( 'NONE',  ( 38.32696717412664356, -286.4477840016668324, -257.3580460447529958 ) ) ;
#17282=CARTESIAN_POINT ( 'NONE',  ( -20.59743046470784478, -296.5945001501515321, -342.5083564738381483 ) ) ;
#17283=CARTESIAN_POINT ( 'NONE',  ( 18.33276714831145782, -277.8692702564945876, -322.3879774774844122 ) ) ;
#17284=CARTESIAN_POINT ( 'NONE',  ( 38.43342003731101642, -276.7344543188282842, -259.8051037481508843 ) ) ;
#17285=CARTESIAN_POINT ( 'NONE',  ( -100.5838947601770030, -277.8843166162832858, -306.9239246804433492 ) ) ;
#17286=CARTESIAN_POINT ( 'NONE',  ( -111.9874385977608000, -274.5676579626259013, -267.6010372180072636 ) ) ;
#17287=CARTESIAN_POINT ( 'NONE',  ( 21.80495789753821612, -284.9221397419026971, -224.5168023592966904 ) ) ;
#17288=CARTESIAN_POINT ( 'NONE',  ( -65.13603027350988839, -291.0093331354566430, -341.3669608528520030 ) ) ;
#17289=CARTESIAN_POINT ( 'NONE',  ( 10.48282447417927976, -293.2935075352553440, -325.9222637526256676 ) ) ;
#17290=ORIENTED_EDGE ( 'NONE', *, *, #70497, .F. ) ;
#17292=CARTESIAN_POINT ( 'NONE',  ( 33.97137422211154245, -293.0110402770283144, -254.6019189343419100 ) ) ;
#17293=EDGE_LOOP ( 'NONE', ( #52940, #63550, #80191, #73505 ) ) ;
#17294=CARTESIAN_POINT ( 'NONE',  ( 3.029155595932095046, -289.6036105966744572, -335.6283790457749774 ) ) ;
#17295=CARTESIAN_POINT ( 'NONE',  ( -110.2609086990360083, -279.2716149022717786, -265.1956858301158491 ) ) ;
#17296=CARTESIAN_POINT ( 'NONE',  ( -106.2296086547079739, -295.9070403498156452, -236.6572818849101623 ) ) ;
#17297=CARTESIAN_POINT ( 'NONE',  ( 14.17243384388611638, -287.4044519914698412, -213.1967195512843318 ) ) ;
#17298=CARTESIAN_POINT ( 'NONE',  ( 39.68137774207683321, -287.9002644426528832, -271.5467260053712266 ) ) ;
#17299=CARTESIAN_POINT ( 'NONE',  ( -105.5862007463691583, -285.2321602334261570, -244.3846743830534933 ) ) ;
#17300=CARTESIAN_POINT ( 'NONE',  ( 64.61140586824606658, 48.03908741837865648, -318.8617120424071345 ) ) ;
#17301=CARTESIAN_POINT ( 'NONE',  ( 152.0371421904949898, 206.9602274457216140, -216.0695842911233342 ) ) ;
#17302=CARTESIAN_POINT ( 'NONE',  ( 188.1653916184831985, 268.5676892509308118, -137.5199885634606005 ) ) ;
#17303=CARTESIAN_POINT ( 'NONE',  ( -74.10323679174986466, -276.7513667766365870, -333.6160873461321330 ) ) ;
#17304=CARTESIAN_POINT ( 'NONE',  ( -107.4161531682840973, -277.1864005470471852, -292.0671586347614266 ) ) ;
#17305=CARTESIAN_POINT ( 'NONE',  ( 53.50357903997114306, -298.6686332334738267, -193.4299620268588740 ) ) ;
#17306=CARTESIAN_POINT ( 'NONE',  ( -37.71430735586704941, -140.7961144971097838, -361.8212181249343757 ) ) ;
#17307=CARTESIAN_POINT ( 'NONE',  ( -6.787134126971194448, -275.3442443828581077, -340.5159738421589850 ) ) ;
#17310=CARTESIAN_POINT ( 'NONE',  ( -110.3985106707871040, -291.0335470360811883, -271.1923067597078330 ) ) ;
#17311=CARTESIAN_POINT ( 'NONE',  ( -36.90828264224272459, -298.8602770830073609, -193.5225356378665538 ) ) ;
#17312=CARTESIAN_POINT ( 'NONE',  ( 33.87054648191396211, -285.9981849473351190, -252.1427390963366690 ) ) ;
#17313=CARTESIAN_POINT ( 'NONE',  ( -106.7547775772333125, -273.6283590829956438, -237.2682567386859205 ) ) ;
#17314=CARTESIAN_POINT ( 'NONE',  ( 10.29312531376072037, -294.5396583741396626, -325.6776924391340344 ) ) ;
#17315=ORIENTED_EDGE ( 'NONE', *, *, #18614, .F. ) ;
#17318=CARTESIAN_POINT ( 'NONE',  ( -88.22403272715123990, -279.6782952476348214, -326.2207852301311846 ) ) ;
#17319=CARTESIAN_POINT ( 'NONE',  ( 29.70519285336511217, -281.5510723694352464, -308.2088008696974839 ) ) ;
#17321=CARTESIAN_POINT ( 'NONE',  ( -110.2096938671491273, -279.5204610175326820, -278.8391610750215364 ) ) ;
#17322=CARTESIAN_POINT ( 'NONE',  ( 28.23292922482151823, -277.8186542418793010, -308.7530702280602100 ) ) ;
#17323=CARTESIAN_POINT ( 'NONE',  ( -110.8792132449868006, -271.1041387173808062, -264.8424321276107207 ) ) ;
#17325=CARTESIAN_POINT ( 'NONE',  ( -100.8128535064753351, -279.2127159221628290, -234.2998826556250265 ) ) ;
#17326=CARTESIAN_POINT ( 'NONE',  ( -35.53784720795390228, -274.8770435820706552, -193.5306673363320158 ) ) ;
#17328=CARTESIAN_POINT ( 'NONE',  ( -2.043237557616166100, -287.2794484643570740, -338.2383366514214345 ) ) ;
#17329=CARTESIAN_POINT ( 'NONE',  ( -65.50058040811698845, -275.6841838574832764, -200.8341629001307638 ) ) ;
#17330=CARTESIAN_POINT ( 'NONE',  ( 35.49543667650704748, -274.4194024630090212, -293.4556583519470792 ) ) ;
#17332=CARTESIAN_POINT ( 'NONE',  ( -110.4986279574996075, -289.7385756856916146, -271.1769837689780616 ) ) ;
#17333=CARTESIAN_POINT ( 'NONE',  ( -68.45190604978013482, -285.0026387793832328, -200.0227409260162972 ) ) ;
#17334=CARTESIAN_POINT ( 'NONE',  ( 18.35280545869903435, -280.4780349904306149, -319.1063337730138869 ) ) ;
#17335=CARTESIAN_POINT ( 'NONE',  ( 21.46995819204322231, -280.7432844575790796, -314.6149968204221636 ) ) ;
#17336=CARTESIAN_POINT ( 'NONE',  ( -22.14238133598405511, -284.3280492697555246, -197.4364398687798712 ) ) ;
#17337=CARTESIAN_POINT ( 'NONE',  ( -57.18235084095585563, -291.3081638130456668, -342.7422772900183645 ) ) ;
#17338=CARTESIAN_POINT ( 'NONE',  ( 28.12868111699887308, -282.3078411552432385, -237.0707713852813754 ) ) ;
#17339=CARTESIAN_POINT ( 'NONE',  ( -111.0966513668062987, -270.7302858448049392, -256.4752353820961162 ) ) ;
#17340=CARTESIAN_POINT ( 'NONE',  ( -21.90813622569987018, -281.2574288904340278, -344.9817955370863842 ) ) ;
#17341=CARTESIAN_POINT ( 'NONE',  ( 37.44480028843214825, -295.4797054385879846, -264.7060316005111531 ) ) ;
#17342=CARTESIAN_POINT ( 'NONE',  ( -50.73866334289159141, -278.1231293446849691, -195.5647585248190126 ) ) ;
#17343=CARTESIAN_POINT ( 'NONE',  ( -80.48787350135009433, -285.6351848300802203, -331.9746990533922144 ) ) ;
#17345=CARTESIAN_POINT ( 'NONE',  ( 0.9488755633414936996, -294.4786119038654988, -205.1618984093132383 ) ) ;
#17346=CARTESIAN_POINT ( 'NONE',  ( 33.97122977329271265, -273.2500782435105862, -246.9674522928405054 ) ) ;
#17347=CARTESIAN_POINT ( 'NONE',  ( 39.54074170339981720, -286.7643335073328217, -271.5589967052943052 ) ) ;
#17348=CARTESIAN_POINT ( 'NONE',  ( -86.44629943036402153, -289.7569767129008369, -215.1998949706504618 ) ) ;
#17350=CARTESIAN_POINT ( 'NONE',  ( 30.72850444077189636, -274.6072431817221400, -298.2036865914383839 ) ) ;
#17351=CARTESIAN_POINT ( 'NONE',  ( -12.61884051280087071, -292.8669864717097653, -340.4127388891209307 ) ) ;
#17352=CARTESIAN_POINT ( 'NONE',  ( -90.94102016010253919, -291.1478831444605362, -320.7181809395301570 ) ) ;
#17354=CARTESIAN_POINT ( 'NONE',  ( 104.1717476309105166, -299.5541904835127980, -195.3611179825600175 ) ) ;
#17355=CARTESIAN_POINT ( 'NONE',  ( 33.82329035037079024, -291.6783760850907470, -242.6786271492420894 ) ) ;
#17356=CARTESIAN_POINT ( 'NONE',  ( -25.02818243234750284, -287.8117877235282549, -197.5437615274489076 ) ) ;
#17357=CARTESIAN_POINT ( 'NONE',  ( -45.93375120771811027, -287.3993972179886782, -345.9128883804920065 ) ) ;
#17358=CARTESIAN_POINT ( 'NONE',  ( 19.96268232578134416, -288.3296445726543880, -224.1720922405726242 ) ) ;
#17360=CARTESIAN_POINT ( 'NONE',  ( 30.63900943890631012, -288.7176255493006352, -297.5389725819040336 ) ) ;
#17362=CARTESIAN_POINT ( 'NONE',  ( -50.16233512675388084, -297.1947526626561285, -344.6704779160114072 ) ) ;
#17364=CARTESIAN_POINT ( 'NONE',  ( -33.76131852421374901, -287.3013387875780609, -193.8419074089113110 ) ) ;
#17365=CARTESIAN_POINT ( 'NONE',  ( -38.54697923533018411, -275.1470060928124326, -345.9115084783269367 ) ) ;
#17366=CARTESIAN_POINT ( 'NONE',  ( -104.9549896037654690, -278.4090899085048818, -307.1604029989917990 ) ) ;
#17367=CARTESIAN_POINT ( 'NONE',  ( 21.95713398562930863, -280.5588514336336061, -221.2755542760304763 ) ) ;
#17368=CARTESIAN_POINT ( 'NONE',  ( -111.7817001273665340, -274.4719972231438874, -270.3855101330484558 ) ) ;
#17369=CARTESIAN_POINT ( 'NONE',  ( -55.20876260339449004, -283.8223120539859110, -197.4666836907997265 ) ) ;
#17371=CARTESIAN_POINT ( 'NONE',  ( 18.91583923652932597, -279.0132568130363211, -221.9065400194043605 ) ) ;
#17372=CARTESIAN_POINT ( 'NONE',  ( 32.71013882639473280, -279.9002235033647139, -297.1517974412815875 ) ) ;
#17374=CARTESIAN_POINT ( 'NONE',  ( 10.07989956661196729, -274.8922012460616315, -330.2106776633971776 ) ) ;
#17375=CARTESIAN_POINT ( 'NONE',  ( -110.9055404474918305, -298.1293450798474396, -265.9942943827450108 ) ) ;
#17376=CARTESIAN_POINT ( 'NONE',  ( 15.53044193640267423, -281.2454830924386897, -325.9131575730608006 ) ) ;
#17377=CARTESIAN_POINT ( 'NONE',  ( -92.02855128315889033, -298.1876951188758085, -221.6501668604090867 ) ) ;
#17378=CARTESIAN_POINT ( 'NONE',  ( -75.54825422226015519, -298.8691424917408881, -204.0163945042463638 ) ) ;
#17379=CARTESIAN_POINT ( 'NONE',  ( 9.501894560030693881, -274.3835815511989153, -214.2791420062029601 ) ) ;
#17380=CARTESIAN_POINT ( 'NONE',  ( 12.23425376785284691, -294.7417573533030577, -214.0137313260702285 ) ) ;
#17381=CARTESIAN_POINT ( 'NONE',  ( 34.85349275685213399, -287.3803270298765256, -243.5869862729987290 ) ) ;
#17382=CARTESIAN_POINT ( 'NONE',  ( -97.41631948712981171, -277.2548627894911988, -224.5104268710522888 ) ) ;
#17384=CARTESIAN_POINT ( 'NONE',  ( -113.3603913257561118, -290.2322206120939541, -282.6150395224028671 ) ) ;
#17387=CARTESIAN_POINT ( 'NONE',  ( 18.84998463886424602, -285.9462176970576479, -223.3745348976965488 ) ) ;
#17388=CARTESIAN_POINT ( 'NONE',  ( -28.07039215829282597, -290.1695408240248071, -195.8840855177694209 ) ) ;
#17390=CARTESIAN_POINT ( 'NONE',  ( -113.2098679957031493, -271.2709011634024137, -296.4525692007673570 ) ) ;
#17391=CARTESIAN_POINT ( 'NONE',  ( 33.75952855361387606, -287.2813925079688033, -287.1719395516581130 ) ) ;
#17393=CARTESIAN_POINT ( 'NONE',  ( -112.9032018303532823, -285.3199108162264679, -284.1908079601929558 ) ) ;
#17394=CARTESIAN_POINT ( 'NONE',  ( 17.33047449263798612, -291.8679161439345080, -216.3995816595989083 ) ) ;
#17395=CARTESIAN_POINT ( 'NONE',  ( 27.42489549581026864, -282.3294860345162647, -229.5361227191907574 ) ) ;
#17396=CARTESIAN_POINT ( 'NONE',  ( -70.21682618138015641, -283.3311927541809609, -335.5535141087693205 ) ) ;
#17397=CARTESIAN_POINT ( 'NONE',  ( -99.09243925907853168, -297.1641952792186885, -224.3407836498434165 ) ) ;
#17398=CARTESIAN_POINT ( 'NONE',  ( -31.31585938465800112, -275.4449934751644378, -197.1026819448701701 ) ) ;
#17399=CARTESIAN_POINT ( 'NONE',  ( -41.66341245129767401, -290.0176888039568439, -195.7905555449135022 ) ) ;
#17401=CARTESIAN_POINT ( 'NONE',  ( -24.51202229943083921, -273.0143260533575926, -198.0421738022632496 ) ) ;
#17404=CARTESIAN_POINT ( 'NONE',  ( -35.93020660818435630, -287.9901466074219911, -195.9344971594413209 ) ) ;
#17405=CARTESIAN_POINT ( 'NONE',  ( -16.57730310165831256, -295.8697747746049345, -344.2424982707772187 ) ) ;
#17406=CARTESIAN_POINT ( 'NONE',  ( -109.7143091425620582, -285.3392583229757520, -260.0607232007880043 ) ) ;
#17407=CARTESIAN_POINT ( 'NONE',  ( 39.47182112341977955, -274.6211883752372955, -271.1811299742585675 ) ) ;
#17408=CARTESIAN_POINT ( 'NONE',  ( 19.33491743841234722, -293.4955389560321919, -218.3892620616566944 ) ) ;
#17409=CARTESIAN_POINT ( 'NONE',  ( 27.65135217505240561, -285.1745211976586347, -231.3213609079857918 ) ) ;
#17410=CARTESIAN_POINT ( 'NONE',  ( 8.896842877848062159, -294.7703685697233595, -331.9057475787039380 ) ) ;
#17411=CARTESIAN_POINT ( 'NONE',  ( -108.3699965399736698, -290.6619709388741057, -287.3042167456861762 ) ) ;
#17414=CARTESIAN_POINT ( 'NONE',  ( -60.31974984533258777, -287.2797680917233833, -197.5412312525447476 ) ) ;
#17415=CARTESIAN_POINT ( 'NONE',  ( -37.30987171927208834, -271.5523547857346784, -190.3611179825600175 ) ) ;
#17417=CARTESIAN_POINT ( 'NONE',  ( -66.69592087417289861, -282.3662966608265492, -337.5503074108665373 ) ) ;
#17418=CARTESIAN_POINT ( 'NONE',  ( -97.04068790367236375, -277.5663565828650121, -318.9798592174279861 ) ) ;
#17419=CARTESIAN_POINT ( 'NONE',  ( 21.95335797599150496, -282.9252805374165973, -224.6880888030420067 ) ) ;
#17420=CARTESIAN_POINT ( 'NONE',  ( -29.05393780148455107, -125.5975973158746939, -363.1324652132601045 ) ) ;
#17421=CARTESIAN_POINT ( 'NONE',  ( -52.81616487699096751, -281.8213018474361320, -345.2426454896730661 ) ) ;
#17422=CARTESIAN_POINT ( 'NONE',  ( 16.22705510898434511, -284.8372971622442265, -218.3780893619775156 ) ) ;
#17423=CARTESIAN_POINT ( 'NONE',  ( 18.43902994631035952, -300.5015369122558013, -194.3579889076426355 ) ) ;
#17424=CARTESIAN_POINT ( 'NONE',  ( -80.18579986607710453, -296.1425222528308723, -329.5419557522594687 ) ) ;
#17426=CARTESIAN_POINT ( 'NONE',  ( -44.33053900005747039, -290.6468708636233487, -197.1498615812441813 ) ) ;
#17427=CARTESIAN_POINT ( 'NONE',  ( -113.9767765952946945, -279.1162914832361253, -277.3301055722702699 ) ) ;
#17428=CARTESIAN_POINT ( 'NONE',  ( 32.06181328548421305, -275.2499161837557153, -247.5677234965944535 ) ) ;
#17429=CARTESIAN_POINT ( 'NONE',  ( 16.72750232955500493, -275.2251956535507702, -324.8228837448914419 ) ) ;
#17431=CARTESIAN_POINT ( 'NONE',  ( -27.99891104009856235, -272.1704639728073971, -195.8940181553785465 ) ) ;
#17432=CARTESIAN_POINT ( 'NONE',  ( -39.07613178564673007, -296.4987845210786759, -346.7522041218230129 ) ) ;
#17435=CARTESIAN_POINT ( 'NONE',  ( -95.35264803199918049, -285.0031781335119945, -315.2029835891626135 ) ) ;
#17436=CARTESIAN_POINT ( 'NONE',  ( -97.23172872720684268, -285.6790394460022640, -317.1281842972056211 ) ) ;
#17437=CARTESIAN_POINT ( 'NONE',  ( -80.69324594591869015, -283.0061209662997044, -329.2844126287917561 ) ) ;
#17438=CARTESIAN_POINT ( 'NONE',  ( -7.199346675504460613, -275.0498768496129287, -337.7248986464228437 ) ) ;
#17439=CARTESIAN_POINT ( 'NONE',  ( -3.029751930673151517, -284.4542661378049502, -336.2051097402604114 ) ) ;
#17440=CARTESIAN_POINT ( 'NONE',  ( -108.4947006497384763, -276.7810372259582437, -289.5433563956704575 ) ) ;
#17441=CARTESIAN_POINT ( 'NONE',  ( 19.42966961143937255, -277.2859519677858771, -316.7623405887259764 ) ) ;
#17443=CARTESIAN_POINT ( 'NONE',  ( -106.0358127635873871, -279.8000975799142793, -235.8147225526070088 ) ) ;
#17444=CARTESIAN_POINT ( 'NONE',  ( -41.01173716849114470, -280.4995061011442203, -193.4970532098554088 ) ) ;
#17445=VERTEX_POINT ( 'NONE', #8604 ) ;
#17447=CARTESIAN_POINT ( 'NONE',  ( 35.95555826579214909, -289.6565411443053222, -289.5396840117884949 ) ) ;
#17449=CARTESIAN_POINT ( 'NONE',  ( -108.6320850499026562, -295.9657148304178804, -253.9208398440649432 ) ) ;
#17450=CARTESIAN_POINT ( 'NONE',  ( -103.1243386839901177, -290.4223665898716717, -230.4343924258889160 ) ) ;
#17451=CARTESIAN_POINT ( 'NONE',  ( 36.56597276341372549, -285.7293118389002871, -265.5427631288117141 ) ) ;
#17452=CARTESIAN_POINT ( 'NONE',  ( 5.079731740519486394, -285.2126242096164788, -210.1672529268174117 ) ) ;
#17453=CARTESIAN_POINT ( 'NONE',  ( -104.9828017033906633, -288.3916052706242681, -300.5319968872909726 ) ) ;
#17454=CARTESIAN_POINT ( 'NONE',  ( -10.61962907896915631, -287.6137106452035823, -201.9877259235813369 ) ) ;
#17455=CARTESIAN_POINT ( 'NONE',  ( -105.7622911574838724, -276.1477636316831195, -301.2060395054491551 ) ) ;
#17456=CARTESIAN_POINT ( 'NONE',  ( 2.741799994701370924, -286.9242427873922452, -335.2285111532752921 ) ) ;
#17457=CARTESIAN_POINT ( 'NONE',  ( 28.36672737334033201, -289.0702739995776369, -234.0953939819645768 ) ) ;
#17458=CARTESIAN_POINT ( 'NONE',  ( 13.34812564381097566, -286.3453118897524519, -325.9345112661461030 ) ) ;
#17459=CARTESIAN_POINT ( 'NONE',  ( -4.711594718966118478, -283.5526203182462837, -335.9254731602548532 ) ) ;
#17460=CARTESIAN_POINT ( 'NONE',  ( -109.4800393152221432, -292.8236813707837314, -249.2403119589064033 ) ) ;
#17463=CARTESIAN_POINT ( 'NONE',  ( -112.3483424243524524, -298.5886378315103116, -261.2332590518147981 ) ) ;
#17464=CARTESIAN_POINT ( 'NONE',  ( -22.15091938936496518, -279.4487684361694733, -198.7420997981078870 ) ) ;
#17465=CARTESIAN_POINT ( 'NONE',  ( 22.59322928371074113, -280.1684892195593193, -315.4689691595826275 ) ) ;
#17466=CARTESIAN_POINT ( 'NONE',  ( 17.43923545849672863, -293.4913175282214866, -324.3182100686868239 ) ) ;
#17467=CARTESIAN_POINT ( 'NONE',  ( -84.57134656037391096, -295.7892314662637432, -213.5863795484178809 ) ) ;
#17468=CARTESIAN_POINT ( 'NONE',  ( 35.52398691814099152, -280.1064382329424234, -260.3990408057631498 ) ) ;
#17469=CARTESIAN_POINT ( 'NONE',  ( 33.43850124423435233, -273.3300717607625074, -247.1413374894281105 ) ) ;
#17470=CARTESIAN_POINT ( 'NONE',  ( -55.91185261690477404, -296.6113598862893923, -341.5221698142247533 ) ) ;
#17472=CARTESIAN_POINT ( 'NONE',  ( -36.53015085399769646, -296.5420233074727889, -194.0546518089647634 ) ) ;
#17473=CARTESIAN_POINT ( 'NONE',  ( 12.71127048530909853, -292.6055182704702133, -327.6031832661492444 ) ) ;
#17474=CARTESIAN_POINT ( 'NONE',  ( 7.017093579273952386, -294.0950555991188935, -211.6442350926261327 ) ) ;
#17476=CARTESIAN_POINT ( 'NONE',  ( 32.90808573650183178, -294.6252299198634432, -290.8406812693814913 ) ) ;
#17478=CARTESIAN_POINT ( 'NONE',  ( -65.97512147630251889, -281.4450370303358113, -340.0781880884891848 ) ) ;
#17479=CARTESIAN_POINT ( 'NONE',  ( 29.49005693663191252, -293.9472564303571289, -299.7297449106809495 ) ) ;
#17480=CARTESIAN_POINT ( 'NONE',  ( 26.72188612836074029, -282.1144386810832998, -313.0794620043430427 ) ) ;
#17481=CARTESIAN_POINT ( 'NONE',  ( 0.6287828212901023228, -282.4739372254828709, -204.9750190359183080 ) ) ;
#17482=CARTESIAN_POINT ( 'NONE',  ( -9.997500605309646460, -286.0661833940826568, -198.3457388481283203 ) ) ;
#17483=CARTESIAN_POINT ( 'NONE',  ( -69.79007302455002559, -289.6238236234000283, -202.9145480600821543 ) ) ;
#17484=CARTESIAN_POINT ( 'NONE',  ( 38.92620833365420197, -280.0627212286973418, -272.7929670375329465 ) ) ;
#17485=CARTESIAN_POINT ( 'NONE',  ( 23.03556061290170476, -287.1073233994362113, -317.6694546320412087 ) ) ;
#17487=CARTESIAN_POINT ( 'NONE',  ( -78.37784092801625491, -297.2142509949216560, -331.7618536361208612 ) ) ;
#17488=CARTESIAN_POINT ( 'NONE',  ( 31.33373573036174520, -277.4122267762397200, -303.9823026842777267 ) ) ;
#17489=CARTESIAN_POINT ( 'NONE',  ( 38.01220734520700262, -291.5360035164656551, -267.5242249225218529 ) ) ;
#17490=CARTESIAN_POINT ( 'NONE',  ( -7.987051889962353712, -280.1143254664593201, -203.4864502092059411 ) ) ;
#17491=CARTESIAN_POINT ( 'NONE',  ( -4.606071721740135239, -292.6383004410208173, -200.6662212011133875 ) ) ;
#17492=CARTESIAN_POINT ( 'NONE',  ( -104.1472886334710211, -283.0978109061526879, -234.9457931597620188 ) ) ;
#17493=CARTESIAN_POINT ( 'NONE',  ( -9.918746155033637990, -278.6941960401608753, -340.1678672598071103 ) ) ;
#17494=CARTESIAN_POINT ( 'NONE',  ( 10.43599032618497979, -293.4319046665373207, -325.8651785753781951 ) ) ;
#17495=CARTESIAN_POINT ( 'NONE',  ( -34.12766851902003395, -296.0922285863567254, -195.3622050365462997 ) ) ;
#17498=CARTESIAN_POINT ( 'NONE',  ( -109.8941877590768712, -280.7584839853464018, -252.8116637138289491 ) ) ;
#17499=CARTESIAN_POINT ( 'NONE',  ( 34.54484983433269463, -292.8868745628288934, -257.2411398688824420 ) ) ;
#17501=CARTESIAN_POINT ( 'NONE',  ( -37.30987171927208834, -295.5523547857347353, -200.3611179825600459 ) ) ;
#17502=CARTESIAN_POINT ( 'NONE',  ( -51.74467765753521320, -296.9310961366714992, -194.9055242722224079 ) ) ;
#17503=CARTESIAN_POINT ( 'NONE',  ( 16.35186851445192247, -289.6243635113345931, -324.9352531123055883 ) ) ;
#17504=CARTESIAN_POINT ( 'NONE',  ( 3.612852318004160956, -288.3177486632435489, -330.8515715501690693 ) ) ;
#17505=CARTESIAN_POINT ( 'NONE',  ( -51.98387877882040442, -281.3816212681724664, -198.0848371837162745 ) ) ;
#17506=CARTESIAN_POINT ( 'NONE',  ( -92.61639579301298397, -299.0064520846261189, -221.1403699812744605 ) ) ;
#17508=CARTESIAN_POINT ( 'NONE',  ( -92.49673606005032411, -278.0347397038505051, -221.9162614387430210 ) ) ;
#17510=CARTESIAN_POINT ( 'NONE',  ( 99.14367289792072313, -299.3839090181289748, -193.3896128337344464 ) ) ;
#17511=CARTESIAN_POINT ( 'NONE',  ( -4.213781257199535446, -294.4124272079877755, -203.6846733922491524 ) ) ;
#17512=CARTESIAN_POINT ( 'NONE',  ( 37.29121272633503992, -295.3465699402026985, -285.7354061505645291 ) ) ;
#17515=CARTESIAN_POINT ( 'NONE',  ( -108.4476387076542210, -290.9800514709121444, -287.3269120187252952 ) ) ;
#17518=CARTESIAN_POINT ( 'NONE',  ( -1.369095648345087568, -290.6636434989744657, -203.6807069975050410 ) ) ;
#17519=CARTESIAN_POINT ( 'NONE',  ( -110.4032385894416564, -272.0598842017238894, -270.3548639019163602 ) ) ;
#17522=CARTESIAN_POINT ( 'NONE',  ( -95.84689571780667450, -291.4067589979324566, -319.3696406983293627 ) ) ;
#17523=CARTESIAN_POINT ( 'NONE',  ( -88.47809603358389552, -298.1948066931273615, -334.5364918783848793 ) ) ;
#17524=CARTESIAN_POINT ( 'NONE',  ( 37.51354006194395652, -289.5249655844303902, -268.2355949849344370 ) ) ;
#17525=CARTESIAN_POINT ( 'NONE',  ( 20.43004431873800897, -272.8944578711617055, -222.7958578237532947 ) ) ;
#17526=CARTESIAN_POINT ( 'NONE',  ( 36.44470349350193317, -277.3449787899690477, -260.5183115621274510 ) ) ;
#17527=CARTESIAN_POINT ( 'NONE',  ( -78.02204385755844385, -289.5805180903799396, -208.0199291073758161 ) ) ;
#17528=CARTESIAN_POINT ( 'NONE',  ( -107.3799877926219466, -280.7857915663868766, -241.4657249381293127 ) ) ;
#17530=CARTESIAN_POINT ( 'NONE',  ( -33.49915127433074957, -282.3511272221823560, -343.3745813227926078 ) ) ;
#17531=CARTESIAN_POINT ( 'NONE',  ( -113.4576900262697166, -279.5088570713479044, -280.1537234041435340 ) ) ;
#17532=CARTESIAN_POINT ( 'NONE',  ( 3.622666666422747372, -279.3847135291584891, -205.5687900262641392 ) ) ;
#17533=CARTESIAN_POINT ( 'NONE',  ( 159.4405072948125053, 218.8499916850896625, -202.6910633192169371 ) ) ;
#17534=CARTESIAN_POINT ( 'NONE',  ( 37.71279890453170935, -276.2904820463264173, -254.1855979908594350 ) ) ;
#17536=CARTESIAN_POINT ( 'NONE',  ( 13.48807720687364053, -276.2682843017167897, -213.3779467923982907 ) ) ;
#17537=CARTESIAN_POINT ( 'NONE',  ( 99.44099354567467230, -302.2645883696979467, -195.3030568020281521 ) ) ;
#17540=CARTESIAN_POINT ( 'NONE',  ( -110.0946008801723224, -291.5134281744877853, -279.3745249762035314 ) ) ;
#17541=CARTESIAN_POINT ( 'NONE',  ( -98.20386861814067458, -291.6986682820609076, -315.8773571623503926 ) ) ;
#17542=CARTESIAN_POINT ( 'NONE',  ( -98.38008394364008780, -290.4589650651858506, -230.0422246006149010 ) ) ;
#17543=CARTESIAN_POINT ( 'NONE',  ( -69.76119187579043057, -285.1443256224156357, -200.5721025084264966 ) ) ;
#17545=CARTESIAN_POINT ( 'NONE',  ( 10.41099691718589071, -280.7803217381434138, -326.6965947874548419 ) ) ;
#17546=CARTESIAN_POINT ( 'NONE',  ( -34.50750544262766795, -290.8767156475494176, -344.5926187316542837 ) ) ;
#17547=CARTESIAN_POINT ( 'NONE',  ( -29.38888906310765137, -281.4296026389145595, -343.6750557052867521 ) ) ;
#17548=CARTESIAN_POINT ( 'NONE',  ( 19.20488162198130055, -282.2057988919751210, -223.3977153338049106 ) ) ;
#17549=CARTESIAN_POINT ( 'NONE',  ( -8.310972920920896456, -289.6224746684585512, -341.4389546749428064 ) ) ;
#17550=CARTESIAN_POINT ( 'NONE',  ( -105.5740067817427956, -279.3947497613974065, -244.0977306108511300 ) ) ;
#17551=CARTESIAN_POINT ( 'NONE',  ( -91.32963113160940338, -288.5940226579364776, -324.7801353660519226 ) ) ;
#17552=CARTESIAN_POINT ( 'NONE',  ( -60.47107579267689204, -286.5625942198196867, -197.0308933975291268 ) ) ;
#17553=CARTESIAN_POINT ( 'NONE',  ( -64.53131373240800883, -286.1989270235665686, -198.3729949387868601 ) ) ;
#17554=CARTESIAN_POINT ( 'NONE',  ( -110.3904050505611991, -284.7115739677781221, -270.9114176497573112 ) ) ;
#17557=CARTESIAN_POINT ( 'NONE',  ( -16.98168619059447693, -294.1727440538232941, -197.3832082391498943 ) ) ;
#17558=CARTESIAN_POINT ( 'NONE',  ( 13.05829143550436733, -293.0504138646471688, -327.9912201096366289 ) ) ;
#17559=CARTESIAN_POINT ( 'NONE',  ( -45.94760717793854354, -276.2225555154175254, -343.1398029587629708 ) ) ;
#17560=CARTESIAN_POINT ( 'NONE',  ( -114.2644733835511914, -295.8744718991156901, -272.4587236071556617 ) ) ;
#17561=CARTESIAN_POINT ( 'NONE',  ( -44.34702231820411811, -290.4419559596660179, -196.9502023754466506 ) ) ;
#17562=CARTESIAN_POINT ( 'NONE',  ( -67.73149879945538032, -293.6963548811190776, -337.8615645571416053 ) ) ;
#17564=CARTESIAN_POINT ( 'NONE',  ( -97.09350757342762961, -292.3505356560202131, -227.6505802757958747 ) ) ;
#17565=CARTESIAN_POINT ( 'NONE',  ( -2.303740420511388720, -293.6070158556617002, -205.9530174245219314 ) ) ;
#17566=CARTESIAN_POINT ( 'NONE',  ( 121.3395553409046528, -299.5541904835127980, -195.3611179825600175 ) ) ;
#17567=CARTESIAN_POINT ( 'NONE',  ( -14.36720165022969375, -292.7547783989718937, -341.9306704774790546 ) ) ;
#17568=CARTESIAN_POINT ( 'NONE',  ( -109.3111139716955194, -298.2784766785204056, -291.6440130419127286 ) ) ;
#17569=CARTESIAN_POINT ( 'NONE',  ( -18.40112929506057426, -289.7434632275808326, -341.1575199974448651 ) ) ;
#17572=CARTESIAN_POINT ( 'NONE',  ( -61.84676131758235584, -279.3488433007075287, -341.6756634153824734 ) ) ;
#17573=CARTESIAN_POINT ( 'NONE',  ( -86.85032266208642682, -276.5178237371862338, -328.8848325797329721 ) ) ;
#17574=CARTESIAN_POINT ( 'NONE',  ( -52.51737664630387314, -273.2113978267725543, -194.9209980936768147 ) ) ;
#17575=CARTESIAN_POINT ( 'NONE',  ( 35.89791776494042352, -279.8051600642812673, -283.7467905870917093 ) ) ;
#17576=CARTESIAN_POINT ( 'NONE',  ( -72.48998852668894699, -275.9093293212183085, -337.9851243546137880 ) ) ;
#17577=CARTESIAN_POINT ( 'NONE',  ( -96.81730069627408852, -294.6366040678423133, -313.5554710507019536 ) ) ;
#17578=CARTESIAN_POINT ( 'NONE',  ( -60.82200480488018002, -275.7477713320995463, -199.0777475753787087 ) ) ;
#17579=CARTESIAN_POINT ( 'NONE',  ( -35.15191628180505745, -298.8830887981370097, -197.1993321852654049 ) ) ;
#17581=CARTESIAN_POINT ( 'NONE',  ( -79.63869437661979589, -287.6403044513306213, -332.7889907146593487 ) ) ;
#17582=CARTESIAN_POINT ( 'NONE',  ( -38.08023040182426655, -273.8759625125530306, -197.3648538482133858 ) ) ;
#17583=CARTESIAN_POINT ( 'NONE',  ( 0.7192939522333362534, -288.5595452132297396, -337.3568675169548783 ) ) ;
#17584=CARTESIAN_POINT ( 'NONE',  ( -98.10055036839052889, -275.1549477452975907, -226.0210668610420157 ) ) ;
#17585=CARTESIAN_POINT ( 'NONE',  ( -110.8416446690041397, -294.7338470644844506, -256.2293286010323641 ) ) ;
#17586=CARTESIAN_POINT ( 'NONE',  ( -92.32534344588422925, -283.0115202022175822, -324.0356723619553350 ) ) ;
#17588=CARTESIAN_POINT ( 'NONE',  ( 24.72548240771276440, -278.9818722485092053, -228.2353968721334354 ) ) ;
#17590=CARTESIAN_POINT ( 'NONE',  ( -79.74767768327657791, -290.2597899866490252, -210.3917056528001694 ) ) ;
#17591=CARTESIAN_POINT ( 'NONE',  ( -23.86409863191952496, -281.0177179328717898, -343.3626230054558732 ) ) ;
#17594=CARTESIAN_POINT ( 'NONE',  ( -108.4599159734351588, -288.8598716074000663, -246.5451564612150719 ) ) ;
#17595=CARTESIAN_POINT ( 'NONE',  ( 17.79151208367478532, -276.3793972487744668, -221.3873016889835128 ) ) ;
#17596=CARTESIAN_POINT ( 'NONE',  ( -47.19003495194347408, -284.3797052228750317, -346.3283413034232012 ) ) ;
#17597=CARTESIAN_POINT ( 'NONE',  ( -93.06643966019032632, -271.3395360653064472, -219.3119560265996597 ) ) ;
#17598=CARTESIAN_POINT ( 'NONE',  ( -69.00916445148507705, -283.4805967386897692, -336.1485608028720549 ) ) ;
#17599=CARTESIAN_POINT ( 'NONE',  ( 34.74539836981070096, -277.1710055054147119, -285.1538577177547609 ) ) ;
#17600=CARTESIAN_POINT ( 'NONE',  ( 29.22873980964546803, -275.9452564596628577, -239.8909788744041975 ) ) ;
#17601=CARTESIAN_POINT ( 'NONE',  ( 5.796042162565585798, -284.4680844852121027, -331.7771934716265605 ) ) ;
#17603=CARTESIAN_POINT ( 'NONE',  ( 204.2968234959853930, 292.4580586366143962, -53.99999999999221956 ) ) ;
#17604=CARTESIAN_POINT ( 'NONE',  ( -33.43696022384644095, -294.8376238862369405, -347.2751672175621138 ) ) ;
#17605=CARTESIAN_POINT ( 'NONE',  ( -40.05847396863813259, -287.9977322027883133, -195.7657699698966098 ) ) ;
#17607=CARTESIAN_POINT ( 'NONE',  ( -99.86837403722181250, -288.6952119285918457, -220.4570493818173702 ) ) ;
#17608=CARTESIAN_POINT ( 'NONE',  ( -89.11087932520128163, -276.9557470734431490, -327.1423728589171560 ) ) ;
#17609=CARTESIAN_POINT ( 'NONE',  ( -53.20269626787620609, -290.2520618232817355, -195.7761941319945720 ) ) ;
#17610=CARTESIAN_POINT ( 'NONE',  ( -92.04880742444235864, -286.7733887058387836, -220.9116240308455019 ) ) ;
#17611=CARTESIAN_POINT ( 'NONE',  ( -96.06350241333637996, -279.6870949627451637, -315.4135757671613192 ) ) ;
#17612=CARTESIAN_POINT ( 'NONE',  ( -40.80805155351878710, -287.4347538856222286, -193.9772171418615017 ) ) ;
#17613=CARTESIAN_POINT ( 'NONE',  ( 34.89237758625882435, -283.8119169392057870, -290.5412732702028507 ) ) ;
#17614=CARTESIAN_POINT ( 'NONE',  ( 16.95673149184141693, -276.4713462457476112, -325.0311802529481042 ) ) ;
#17615=CARTESIAN_POINT ( 'NONE',  ( -82.54799658096474957, -277.4843043900669386, -332.6940207346409579 ) ) ;
#17616=CARTESIAN_POINT ( 'NONE',  ( -93.85324223422927048, -299.1488582801878238, -221.8878161867566803 ) ) ;
#17618=CARTESIAN_POINT ( 'NONE',  ( 21.31550574532285580, -278.6948066931273615, -317.0979686699210447 ) ) ;
#17619=CARTESIAN_POINT ( 'NONE',  ( -97.24259044483734726, -295.3214412754409750, -223.9484999571485275 ) ) ;
#17621=CARTESIAN_POINT ( 'NONE',  ( -105.3273519283102360, -277.7022816625387804, -297.1181654807863879 ) ) ;
#17622=CARTESIAN_POINT ( 'NONE',  ( -7.857672798845277917, -275.6349315123820816, -199.6033272883307177 ) ) ;
#17623=CARTESIAN_POINT ( 'NONE',  ( 38.02596540867186548, -280.4280202092706418, -255.7825307694277512 ) ) ;
#17624=CARTESIAN_POINT ( 'NONE',  ( 9.656927660583086492, -288.4694223126115844, -213.1850478405015110 ) ) ;
#17625=CARTESIAN_POINT ( 'NONE',  ( -94.12259327859879932, -297.3741066089525020, -321.3574167657899920 ) ) ;
#17626=CARTESIAN_POINT ( 'NONE',  ( -70.62141972905970988, -296.6862643438914233, -339.3717040882862079 ) ) ;
#17627=CARTESIAN_POINT ( 'NONE',  ( -50.02387512309542217, -293.8902599616650377, -196.5576308607510896 ) ) ;
#17628=CARTESIAN_POINT ( 'NONE',  ( 21.98458729161788483, -278.9256080531673661, -224.7286594058828371 ) ) ;
#17629=CARTESIAN_POINT ( 'NONE',  ( 10.17734072955849811, -282.6330770578432521, -212.9942484425526743 ) ) ;
#17630=CARTESIAN_POINT ( 'NONE',  ( -95.56257679745787925, -295.2744248083453726, -223.9753041816722146 ) ) ;
#17631=CARTESIAN_POINT ( 'NONE',  ( -111.0954516566918215, -285.9094528261143751, -289.5654579535222410 ) ) ;
#17633=CARTESIAN_POINT ( 'NONE',  ( 29.09586790816225843, -286.0558130400837626, -239.3728036355984727 ) ) ;
#17634=CARTESIAN_POINT ( 'NONE',  ( 6.133466362344496936, -279.9740074315837433, -206.9322390316848157 ) ) ;
#17635=CARTESIAN_POINT ( 'NONE',  ( -29.32149395268238479, -125.4031318350040891, -363.7124165658669881 ) ) ;
#17637=CARTESIAN_POINT ( 'NONE',  ( 32.69145310020566342, -286.9448490079262797, -249.6422584931054018 ) ) ;
#17639=CARTESIAN_POINT ( 'NONE',  ( -96.02487318110094350, -284.9640772687168919, -319.7552888296561946 ) ) ;
#17640=CARTESIAN_POINT ( 'NONE',  ( 7.340503886933810840, -275.0141102195086091, -212.6065672437735543 ) ) ;
#17641=CARTESIAN_POINT ( 'NONE',  ( -49.26769202525431979, -284.6984497089737829, -194.6387801587113415 ) ) ;
#17642=CARTESIAN_POINT ( 'NONE',  ( -73.27665556041465322, -290.5073833521827851, -202.5954748960363645 ) ) ;
#17643=CARTESIAN_POINT ( 'NONE',  ( 12.82931170852911507, -281.6738949897509769, -212.2604313806997425 ) ) ;
#17645=CARTESIAN_POINT ( 'NONE',  ( -40.99474559807290319, -281.5271148272101414, -194.1288639248617471 ) ) ;
#17646=CARTESIAN_POINT ( 'NONE',  ( 39.68926002210008619, -281.8799913415469405, -269.9261499705065148 ) ) ;
#17647=CARTESIAN_POINT ( 'NONE',  ( -102.0455923789670294, -287.6237833571632905, -301.4846348637937581 ) ) ;
#17648=CARTESIAN_POINT ( 'NONE',  ( -103.8349779299932152, -256.5568498903555792, -326.8183980474310601 ) ) ;
#17650=CARTESIAN_POINT ( 'NONE',  ( 33.84996063021831958, -277.8507559610383169, -293.4213839146042346 ) ) ;
#17651=CARTESIAN_POINT ( 'NONE',  ( -110.7306624032010802, -265.9561541865978143, -306.7379753279722081 ) ) ;
#17652=CARTESIAN_POINT ( 'NONE',  ( 35.95402134271872541, -279.3891321913799288, -256.1662435223460079 ) ) ;
#17653=CARTESIAN_POINT ( 'NONE',  ( -72.88920365406468704, -296.9164125769060547, -206.4841451252907234 ) ) ;
#17654=CARTESIAN_POINT ( 'NONE',  ( -70.86523179119832605, -291.1293228829475197, -201.1101271706874627 ) ) ;
#17656=CARTESIAN_POINT ( 'NONE',  ( -65.30930134969403866, -296.2685389482138589, -199.1960651998306275 ) ) ;
#17657=CARTESIAN_POINT ( 'NONE',  ( 20.98531840833684470, -285.3221071166516367, -225.1460836898898492 ) ) ;
#17658=CARTESIAN_POINT ( 'NONE',  ( 22.33329217630785024, -296.0213409799287660, -314.5172135519637209 ) ) ;
#17659=CARTESIAN_POINT ( 'NONE',  ( -71.42167675060044019, -286.9072998483213155, -205.2473815473493630 ) ) ;
#17661=CARTESIAN_POINT ( 'NONE',  ( 27.91225365938942815, -295.0249063270122178, -310.8929476730986039 ) ) ;
#17662=CARTESIAN_POINT ( 'NONE',  ( -108.1513204925075655, -284.8071272311215125, -288.3607320252058912 ) ) ;
#17663=CARTESIAN_POINT ( 'NONE',  ( -46.06932200116946063, -296.7387178400814491, -194.2569963170201106 ) ) ;
#17664=CARTESIAN_POINT ( 'NONE',  ( 20.25086708675662805, -293.6645410333546806, -219.4761759203548195 ) ) ;
#17665=CARTESIAN_POINT ( 'NONE',  ( -103.1664468090598774, -291.5659427370477488, -230.4258660393881826 ) ) ;
#17666=CARTESIAN_POINT ( 'NONE',  ( -61.25300888706676972, -289.5381760259506336, -339.3339337720379945 ) ) ;
#17669=CARTESIAN_POINT ( 'NONE',  ( -51.59190099714205502, -299.7323131751791152, -195.8950322800952506 ) ) ;
#17670=CARTESIAN_POINT ( 'NONE',  ( -91.87556230996639783, -272.0898907607852948, -216.5645884134065113 ) ) ;
#17671=CARTESIAN_POINT ( 'NONE',  ( -1.146107736160122847, -281.6178869853226843, -334.0265524014146763 ) ) ;
#17673=CARTESIAN_POINT ( 'NONE',  ( -87.06020940125013396, -277.2304375771291802, -329.1470700126715201 ) ) ;
#17674=CARTESIAN_POINT ( 'NONE',  ( -110.3714176747848370, -271.0953383341310996, -259.3776521411577392 ) ) ;
#17675=CARTESIAN_POINT ( 'NONE',  ( -66.57761392687062596, -281.5255483142537969, -202.1114281615460300 ) ) ;
#17676=CARTESIAN_POINT ( 'NONE',  ( 8.321853300821368649, -274.5596669924367461, -328.9561286365883461 ) ) ;
#17678=CARTESIAN_POINT ( 'NONE',  ( -108.6813437575163448, -297.5301244360953774, -287.6705433096478828 ) ) ;
#17679=CARTESIAN_POINT ( 'NONE',  ( -100.1687726011513035, -298.1505643338160780, -232.4869132194841370 ) ) ;
#17680=CARTESIAN_POINT ( 'NONE',  ( -110.0559311812380798, -298.4435442172528496, -247.4027046910749732 ) ) ;
#17681=CARTESIAN_POINT ( 'NONE',  ( 20.60261249216338442, -272.9102088506251107, -222.1857773883080256 ) ) ;
#17682=CARTESIAN_POINT ( 'NONE',  ( 33.74494510461933316, -293.9783495547694656, -253.2612146701854101 ) ) ;
#17683=CARTESIAN_POINT ( 'NONE',  ( 32.36498716322867608, -291.8141178373648472, -246.6152450996182210 ) ) ;
#17685=CARTESIAN_POINT ( 'NONE',  ( 18.04094024406537855, -275.3119379607195469, -216.8778110723447412 ) ) ;
#17687=CARTESIAN_POINT ( 'NONE',  ( -107.1971508084990887, -273.0015397566239130, -248.9932279303020550 ) ) ;
#17689=CARTESIAN_POINT ( 'NONE',  ( -58.36740504657306872, -282.0030912873896796, -343.9772460047602749 ) ) ;
#17691=CARTESIAN_POINT ( 'NONE',  ( -70.29679799779499660, -282.6951431472427885, -335.6940631539447963 ) ) ;
#17692=CARTESIAN_POINT ( 'NONE',  ( -52.57165735092634407, -281.2465061577509573, -344.0219031879252611 ) ) ;
#17693=CARTESIAN_POINT ( 'NONE',  ( 34.70189891626354495, -273.9297394749829664, -255.2963710662131120 ) ) ;
#17694=CARTESIAN_POINT ( 'NONE',  ( 34.96609505648138594, -283.8089800578763970, -290.3229119254758643 ) ) ;
#17697=CARTESIAN_POINT ( 'NONE',  ( -34.11644831687502943, -272.4919584861413568, -194.2294020716536238 ) ) ;
#17698=CARTESIAN_POINT ( 'NONE',  ( -112.3999288486476189, -280.5006066881134643, -274.3972950378903306 ) ) ;
#17700=CARTESIAN_POINT ( 'NONE',  ( -85.17160331915195570, -285.6269433390694417, -328.8556865841721901 ) ) ;
#17702=CARTESIAN_POINT ( 'NONE',  ( -110.3148300015880068, -288.3289346875240540, -287.7336675289198524 ) ) ;
#17704=CARTESIAN_POINT ( 'NONE',  ( -107.9891537345519765, -295.0854200283829982, -290.2625703017852743 ) ) ;
#17705=CARTESIAN_POINT ( 'NONE',  ( -95.93996395916997244, -288.0601211273924491, -315.9569754350310973 ) ) ;
#17706=CARTESIAN_POINT ( 'NONE',  ( -117.0946091816712453, -269.6096274233381109, -270.3236525939013859 ) ) ;
#17707=CARTESIAN_POINT ( 'NONE',  ( -112.0398673256333097, -294.6454663220733892, -263.0808577613462376 ) ) ;
#17708=CARTESIAN_POINT ( 'NONE',  ( 2.798800585097338534, -287.0042363100206444, -335.3187633961321694 ) ) ;
#17709=CARTESIAN_POINT ( 'NONE',  ( 0.7961079936739583474, -282.1697093603694384, -207.1201059404870648 ) ) ;
#17710=CARTESIAN_POINT ( 'NONE',  ( -16.44234836096939389, -281.0256802891428265, -343.4717528126160460 ) ) ;
#17711=CARTESIAN_POINT ( 'NONE',  ( 10.11526302078678619, -288.3766170477246078, -325.8971964888217485 ) ) ;
#17712=CARTESIAN_POINT ( 'NONE',  ( 29.85989559455946818, -283.3794908267593655, -300.4749768059178336 ) ) ;
#17713=CARTESIAN_POINT ( 'NONE',  ( 19.48391776830431610, -283.0057355178621492, -316.4617847527654817 ) ) ;
#17714=CARTESIAN_POINT ( 'NONE',  ( 31.20512715447165064, -289.1217149490772158, -238.9348096278522746 ) ) ;
#17715=CARTESIAN_POINT ( 'NONE',  ( -80.62677572701804252, -297.6498053103783263, -206.6149693722878737 ) ) ;
#17716=CARTESIAN_POINT ( 'NONE',  ( -21.35479054832686430, -274.2517471427060514, -195.0390181572846018 ) ) ;
#17717=CARTESIAN_POINT ( 'NONE',  ( -22.43628846829315648, -294.2238390051361989, -197.2196420411085001 ) ) ;
#17719=CARTESIAN_POINT ( 'NONE',  ( -95.95921662488163406, -280.4090924074130839, -317.1477375740089997 ) ) ;
#17721=CARTESIAN_POINT ( 'NONE',  ( -12.49677587509686383, -274.7297834191364245, -341.3576404100920172 ) ) ;
#17723=CARTESIAN_POINT ( 'NONE',  ( -113.3214010048881875, -295.0334561552160721, -263.9176088293445446 ) ) ;
#17724=CARTESIAN_POINT ( 'NONE',  ( -29.97135204591434743, -273.4964847907365311, -197.6316835197017667 ) ) ;
#17725=CARTESIAN_POINT ( 'NONE',  ( -94.63118473278014164, -291.4227757615917653, -316.7143563632914720 ) ) ;
#17726=CARTESIAN_POINT ( 'NONE',  ( -92.74232247938222429, -292.1736885089243287, -222.4635241837306410 ) ) ;
#17727=CARTESIAN_POINT ( 'NONE',  ( -1.924309616885777841, -284.3364837601328645, -335.3647026359278698 ) ) ;
#17728=CARTESIAN_POINT ( 'NONE',  ( -113.0845722507409903, -292.1093589700644202, -259.8922154418312402 ) ) ;
#17729=CARTESIAN_POINT ( 'NONE',  ( -1.052632141082161077, -293.8387203449771619, -203.0083020189727279 ) ) ;
#17730=CARTESIAN_POINT ( 'NONE',  ( -50.47329019489183111, -295.0578508532300930, -342.1703189724210574 ) ) ;
#17731=CARTESIAN_POINT ( 'NONE',  ( 33.72787448323956028, -289.2424871893406362, -246.4003956917890150 ) ) ;
#17732=CARTESIAN_POINT ( 'NONE',  ( -2.890936421800040179, -282.7762008881508677, -339.2390045673786858 ) ) ;
#17733=CARTESIAN_POINT ( 'NONE',  ( -111.7894443477939319, -294.4636028563085688, -283.5742726090718975 ) ) ;
#17734=CARTESIAN_POINT ( 'NONE',  ( -44.42132949944037534, -282.9725524954667435, -347.0883227273838543 ) ) ;
#17735=CARTESIAN_POINT ( 'NONE',  ( 34.09773391867471304, -277.8127698190616002, -292.0446562364148804 ) ) ;
#17736=CARTESIAN_POINT ( 'NONE',  ( -3.112352779071856812, -284.5041144407283582, -203.6133033453804444 ) ) ;
#17737=CARTESIAN_POINT ( 'NONE',  ( -12.29720411840080097, -274.8695054448504607, -341.9219351106789873 ) ) ;
#17739=CARTESIAN_POINT ( 'NONE',  ( 13.96343427941700632, -281.8163053036024621, -322.4493760913728124 ) ) ;
#17740=CARTESIAN_POINT ( 'NONE',  ( -33.94829648898074481, -281.2990232641605530, -193.8333875115237959 ) ) ;
#17741=CARTESIAN_POINT ( 'NONE',  ( 36.46832320789222592, -286.3435441246020332, -249.0795967653575929 ) ) ;
#17742=CARTESIAN_POINT ( 'NONE',  ( 5.066164061071487978, -294.3939564883672233, -209.6390351055500787 ) ) ;
#17743=CARTESIAN_POINT ( 'NONE',  ( 38.83060425639602187, -277.1263172982480114, -268.3067426007121981 ) ) ;
#17744=CARTESIAN_POINT ( 'NONE',  ( 36.76526535727481360, -277.1067776853337250, -289.3731126372894096 ) ) ;
#17745=CARTESIAN_POINT ( 'NONE',  ( -110.2802261272020274, -278.3459589253014315, -273.3563524575844212 ) ) ;
#17746=CARTESIAN_POINT ( 'NONE',  ( -53.04402875454506727, -299.8507008681648358, -197.1405474645553966 ) ) ;
#17747=CARTESIAN_POINT ( 'NONE',  ( 23.49656973147837391, -284.9568857992414337, -226.6992580576661283 ) ) ;
#17748=CARTESIAN_POINT ( 'NONE',  ( 19.51119775226462849, -293.9253648607297009, -322.3376204120130524 ) ) ;
#17749=CARTESIAN_POINT ( 'NONE',  ( -113.5893940586632027, -292.1411720431717072, -271.2400806128175077 ) ) ;
#17750=CARTESIAN_POINT ( 'NONE',  ( 31.12196087148551982, -292.1239159680870898, -244.1513260037536952 ) ) ;
#17752=CARTESIAN_POINT ( 'NONE',  ( -20.06304599662741239, -291.9469558478332374, -199.3614184540020631 ) ) ;
#17754=CARTESIAN_POINT ( 'NONE',  ( 7.763859992516961128, -289.5322511306217166, -332.4506485357376278 ) ) ;
#17755=CARTESIAN_POINT ( 'NONE',  ( -35.66877213859904572, -280.7250724815806961, -197.2659092102464342 ) ) ;
#17756=CARTESIAN_POINT ( 'NONE',  ( -97.09681548444250154, -296.1193449961528472, -222.2901423307159519 ) ) ;
#17757=CARTESIAN_POINT ( 'NONE',  ( 22.90684029761423801, -287.5630349142196565, -222.5549246932329197 ) ) ;
#17758=CARTESIAN_POINT ( 'NONE',  ( 37.35528158426782852, -287.6526170707588790, -251.7572147712762671 ) ) ;
#17759=CARTESIAN_POINT ( 'NONE',  ( -107.7804260445666102, -284.6306542899195051, -289.6560006776313116 ) ) ;
#17760=CARTESIAN_POINT ( 'NONE',  ( -112.7013083777456330, -271.1594590305112433, -296.3539449067754390 ) ) ;
#17761=CARTESIAN_POINT ( 'NONE',  ( -108.3564486399562412, -260.6790360280811569, -316.7380296206242747 ) ) ;
#17762=CARTESIAN_POINT ( 'NONE',  ( 201.5605854984582663, 292.5235874916616581, -68.22477292250835035 ) ) ;
#17763=CARTESIAN_POINT ( 'NONE',  ( 18.42487748536285608, -275.4212177974885094, -317.7181718254829548 ) ) ;
#17764=CARTESIAN_POINT ( 'NONE',  ( 36.00789036824063061, -274.4887990777709774, -271.6038690425473305 ) ) ;
#17765=CARTESIAN_POINT ( 'NONE',  ( -113.8411827663665576, -272.3261748891251841, -261.7836214039719493 ) ) ;
#17766=CARTESIAN_POINT ( 'NONE',  ( 203.5339397030482189, 292.0436732951557701, -68.28815551792725103 ) ) ;
#17767=CARTESIAN_POINT ( 'NONE',  ( -4.223575908080033692, -275.3095016481788093, -339.3428195689347717 ) ) ;
#17768=CARTESIAN_POINT ( 'NONE',  ( -43.58970876774290559, -275.7324274079122688, -196.5605576942260484 ) ) ;
#17770=CARTESIAN_POINT ( 'NONE',  ( -69.99432313723040977, -289.9866398203401445, -335.7339556616880714 ) ) ;
#17771=CARTESIAN_POINT ( 'NONE',  ( -109.7022403020554577, -297.6819397677380152, -244.5132738567006072 ) ) ;
#17772=CARTESIAN_POINT ( 'NONE',  ( -85.18305597396116013, -297.9037045220665618, -210.1055657580390630 ) ) ;
#17773=CARTESIAN_POINT ( 'NONE',  ( -55.80126008196373988, -295.4630507210210340, -341.0410072046119012 ) ) ;
#17775=CARTESIAN_POINT ( 'NONE',  ( -94.11240937194851597, -279.7846083622071092, -320.2249402561186571 ) ) ;
#17777=CARTESIAN_POINT ( 'NONE',  ( 39.57938809120850721, -281.0185663768605764, -267.0662712064930702 ) ) ;
#17778=CARTESIAN_POINT ( 'NONE',  ( -100.8437493448315934, -279.1304673795540907, -307.0924776408278376 ) ) ;
#17779=CARTESIAN_POINT ( 'NONE',  ( -14.86772463289301527, -278.5251861102902922, -343.0033648326723323 ) ) ;
#17780=CARTESIAN_POINT ( 'NONE',  ( -101.7213526399206103, -295.6101781062986902, -234.7151468470400744 ) ) ;
#17783=CARTESIAN_POINT ( 'NONE',  ( -110.3919245767296502, -278.7151521488672756, -270.6401720130731405 ) ) ;
#17784=CARTESIAN_POINT ( 'NONE',  ( -7.762213384313215059, -275.2327533195534670, -199.3877004573737395 ) ) ;
#17785=CARTESIAN_POINT ( 'NONE',  ( -48.81170910836917898, -287.8800048916109517, -346.0568836833317619 ) ) ;
#17786=CARTESIAN_POINT ( 'NONE',  ( -69.30323031890370089, -275.6318797607426632, -202.4982656123123945 ) ) ;
#17787=CARTESIAN_POINT ( 'NONE',  ( 38.15070460945472774, -274.2799164297738912, -282.5038458828271359 ) ) ;
#17789=CARTESIAN_POINT ( 'NONE',  ( -95.90370837899199330, -289.1348904764423082, -314.2351120136659688 ) ) ;
#17790=CARTESIAN_POINT ( 'NONE',  ( -76.04822907539227117, -284.8982021472038468, -203.8534527296125987 ) ) ;
#17791=CARTESIAN_POINT ( 'NONE',  ( -13.22000077407985685, -280.9744824399166419, -340.3877236193171143 ) ) ;
#17792=CARTESIAN_POINT ( 'NONE',  ( 26.05752155882104404, -280.6371631298986244, -307.8236974248523552 ) ) ;
#17793=CARTESIAN_POINT ( 'NONE',  ( -77.81182374204136920, -283.5842397628268827, -207.8221080490869781 ) ) ;
#17794=CARTESIAN_POINT ( 'NONE',  ( 12.60499006191922788, -290.3565190197821266, -326.3792900967713990 ) ) ;
#17795=CARTESIAN_POINT ( 'NONE',  ( -107.4916046095127200, -279.4707790256399562, -292.1210325950855236 ) ) ;
#17797=CARTESIAN_POINT ( 'NONE',  ( 32.82126330089431576, -280.3358637658288330, -300.2211750137091144 ) ) ;
#17798=CARTESIAN_POINT ( 'NONE',  ( 32.58854498080377482, -295.1980916641944646, -243.1112403593733120 ) ) ;
#17799=CARTESIAN_POINT ( 'NONE',  ( -109.5792601793995118, -277.0944433828132105, -246.6207923682664216 ) ) ;
#17800=CARTESIAN_POINT ( 'NONE',  ( -82.75481009332455073, -285.6710795534855265, -330.3237122468634084 ) ) ;
#17802=CARTESIAN_POINT ( 'NONE',  ( -112.9289674395089378, -292.4970901128252194, -268.4166340671497437 ) ) ;
#17803=CARTESIAN_POINT ( 'NONE',  ( 36.53880701214865212, -286.4819411836165273, -249.0574248363113270 ) ) ;
#17804=CARTESIAN_POINT ( 'NONE',  ( -107.7589061983304788, -289.2420863045257420, -248.2310885533853480 ) ) ;
#17806=CARTESIAN_POINT ( 'NONE',  ( 36.13629455319700412, -274.2174135372637238, -268.8685449644514733 ) ) ;
#17807=CARTESIAN_POINT ( 'NONE',  ( -23.30816682774668891, -293.0105356823012244, -343.3102691443972390 ) ) ;
#17810=CARTESIAN_POINT ( 'NONE',  ( 34.80349393727056651, -291.7140716903027169, -245.3458976984586286 ) ) ;
#17811=CARTESIAN_POINT ( 'NONE',  ( -38.65940762213166693, -287.6355219465610844, -196.5602618129810537 ) ) ;
#17812=CARTESIAN_POINT ( 'NONE',  ( -73.95893579426329723, -287.7714655530916161, -336.9578954560478792 ) ) ;
#17813=CARTESIAN_POINT ( 'NONE',  ( -27.77780136780434006, -287.6012640409599612, -197.3960115495131902 ) ) ;
#17815=CARTESIAN_POINT ( 'NONE',  ( 31.99036457150398505, -288.0453523541719392, -247.0016117508360480 ) ) ;
#17816=CARTESIAN_POINT ( 'NONE',  ( 30.68993463090458462, -295.1061912378903571, -237.8346389110484722 ) ) ;
#17818=CARTESIAN_POINT ( 'NONE',  ( 21.77391092965908825, -288.0992556379646317, -221.6440444926696500 ) ) ;
#17819=CARTESIAN_POINT ( 'NONE',  ( -61.96036808352577197, -275.4494254994771154, -341.8533129174110741 ) ) ;
#17820=CARTESIAN_POINT ( 'NONE',  ( -80.21088674958232900, -277.9483797814314130, -334.3625740726946560 ) ) ;
#17822=CARTESIAN_POINT ( 'NONE',  ( -16.99051278330689740, -290.3927826601469064, -197.5933822124611083 ) ) ;
#17823=CARTESIAN_POINT ( 'NONE',  ( -94.96178988952230782, -279.2441756305032641, -219.2834784924319251 ) ) ;
#17824=CARTESIAN_POINT ( 'NONE',  ( -94.00916981728916255, -299.2085867525287313, -221.7549831944050993 ) ) ;
#17826=CARTESIAN_POINT ( 'NONE',  ( -108.4197741028974349, -282.8633569967754511, -246.2631681985445198 ) ) ;
#17829=CARTESIAN_POINT ( 'NONE',  ( -111.3890742955827022, -276.7601902350255045, -265.0836321121481660 ) ) ;
#17830=CARTESIAN_POINT ( 'NONE',  ( 31.35160356192858444, -279.1578583464187773, -240.2574525251123987 ) ) ;
#17832=CARTESIAN_POINT ( 'NONE',  ( 12.23930627921130920, -274.8563713899467871, -328.3648381615888638 ) ) ;
#17833=CARTESIAN_POINT ( 'NONE',  ( -88.97394391291211946, -297.3136534890559801, -323.0143604032419944 ) ) ;
#17834=CARTESIAN_POINT ( 'NONE',  ( -66.47162356621498702, -282.3451124456813091, -341.3184654210264739 ) ) ;
#17835=CARTESIAN_POINT ( 'NONE',  ( -82.09735401828436352, -298.3662192843175944, -212.3283994760195412 ) ) ;
#17836=CARTESIAN_POINT ( 'NONE',  ( -113.2872878658722300, -297.9837553270439798, -261.1109301218626229 ) ) ;
#17837=CARTESIAN_POINT ( 'NONE',  ( -19.26228503191035202, -273.9578373196731604, -199.5610796301048140 ) ) ;
#17838=CARTESIAN_POINT ( 'NONE',  ( 37.52953047237122775, -295.4854416473697825, -265.1527522131964361 ) ) ;
#17839=CARTESIAN_POINT ( 'NONE',  ( 19.62567604681163402, -288.4230589538124150, -322.1853722743121580 ) ) ;
#17840=CARTESIAN_POINT ( 'NONE',  ( -112.2855505907938181, -276.7597884635018772, -260.3342467771904580 ) ) ;
#17841=CARTESIAN_POINT ( 'NONE',  ( -98.34696146254658800, -291.0126312216229962, -223.3572542702410715 ) ) ;
#17842=CARTESIAN_POINT ( 'NONE',  ( 29.63540557068274595, -287.0097712819272147, -300.1091083374892037 ) ) ;
#17844=CARTESIAN_POINT ( 'NONE',  ( -67.50053590734492559, -289.6564177026513676, -201.6780268868807298 ) ) ;
#17846=CARTESIAN_POINT ( 'NONE',  ( 201.7194887906492795, 294.2213704821156739, -83.28174295417332473 ) ) ;
#17847=CARTESIAN_POINT ( 'NONE',  ( -75.90653936328065754, -289.0901101615197035, -332.4154620398738871 ) ) ;
#17849=CARTESIAN_POINT ( 'NONE',  ( -67.77700842209684140, -284.3831914922274677, -340.8346039365395086 ) ) ;
#17850=CARTESIAN_POINT ( 'NONE',  ( 39.47617173764678000, -292.6104118191377097, -270.3220790589136300 ) ) ;
#17851=CARTESIAN_POINT ( 'NONE',  ( 18.55927979783339765, -282.4394403096026167, -218.5777146674589062 ) ) ;
#17852=CARTESIAN_POINT ( 'NONE',  ( 22.47916806744032669, -282.2244053468974130, -222.6458313036172001 ) ) ;
#17853=CARTESIAN_POINT ( 'NONE',  ( -37.54265456413710211, -282.8880918631435861, -343.3732708148669985 ) ) ;
#17854=CARTESIAN_POINT ( 'NONE',  ( -113.2038780994886338, -296.3834467473143377, -283.8506665897165249 ) ) ;
#17855=CARTESIAN_POINT ( 'NONE',  ( -13.92405418389636651, -275.6776531361581988, -200.6986651414621008 ) ) ;
#17856=CARTESIAN_POINT ( 'NONE',  ( -68.46450504575271623, -289.6613386426316197, -202.5000590882436029 ) ) ;
#17857=CARTESIAN_POINT ( 'NONE',  ( -110.5838718324912691, -271.4191342215616487, -264.8685366628302518 ) ) ;
#17860=CARTESIAN_POINT ( 'NONE',  ( -96.10864961828872310, -287.1038208322881928, -224.6484012227728329 ) ) ;
#17861=CARTESIAN_POINT ( 'NONE',  ( -2.097246812907239910, -295.6762117236767722, -338.4736793880846903 ) ) ;
#17862=CARTESIAN_POINT ( 'NONE',  ( -98.19651279018879109, -285.7650456333064994, -229.8569892538839383 ) ) ;
#17863=CARTESIAN_POINT ( 'NONE',  ( 14.71478924110950892, -275.3993183041594648, -326.8510239473284287 ) ) ;
#17864=CARTESIAN_POINT ( 'NONE',  ( 37.68630615537986017, -294.4153881692369055, -287.2761744134524520 ) ) ;
#17865=CARTESIAN_POINT ( 'NONE',  ( 22.03882654398868013, -285.0516125766982327, -223.2845220377510316 ) ) ;
#17866=CARTESIAN_POINT ( 'NONE',  ( -72.16649807255318194, -291.9375431129384424, -201.6953917857080398 ) ) ;
#17867=CARTESIAN_POINT ( 'NONE',  ( -56.06691911712367471, -289.6332004899992967, -340.9931032738587078 ) ) ;
#17870=CARTESIAN_POINT ( 'NONE',  ( 202.6187423002989760, 291.9839001675061354, -68.23006720443765971 ) ) ;
#17871=CARTESIAN_POINT ( 'NONE',  ( -112.3206975191757664, -286.2545543845835141, -255.9133864947453674 ) ) ;
#17872=CARTESIAN_POINT ( 'NONE',  ( -88.47809603358389552, -276.9094976428775681, -206.1857440867352693 ) ) ;
#17874=CARTESIAN_POINT ( 'NONE',  ( -29.42487889863111761, -281.8699822111988169, -343.2922167462845664 ) ) ;
#17875=CARTESIAN_POINT ( 'NONE',  ( -113.2149299087082710, -278.3814987222999662, -257.3612220517189826 ) ) ;
#17876=CARTESIAN_POINT ( 'NONE',  ( -77.83478494667707537, -281.5074748238621964, -207.3681125572547046 ) ) ;
#17877=CARTESIAN_POINT ( 'NONE',  ( 140.6823888433080185, 178.4315446074800775, -239.9256222415464208 ) ) ;
#17878=CARTESIAN_POINT ( 'NONE',  ( -67.66434415870708108, -282.0170496562066091, -340.4977243517851093 ) ) ;
#17879=CARTESIAN_POINT ( 'NONE',  ( 29.13416963295219375, -285.1198088678092972, -236.2940885028409070 ) ) ;
#17880=CARTESIAN_POINT ( 'NONE',  ( -109.8618611376048761, -274.6944470158696276, -248.2468764230110025 ) ) ;
#17881=CARTESIAN_POINT ( 'NONE',  ( -92.23276838147855017, -296.3567580256465135, -318.5789473383214272 ) ) ;
#17883=CARTESIAN_POINT ( 'NONE',  ( 6.986933163425442572, -291.3550503286494404, -211.7418741532002002 ) ) ;
#17884=CARTESIAN_POINT ( 'NONE',  ( -34.28682982873007035, -277.6660963884695548, -347.1984822937913577 ) ) ;
#17885=CARTESIAN_POINT ( 'NONE',  ( -40.77494098136474321, -274.0079063102132864, -197.3921958657863343 ) ) ;
#17886=CARTESIAN_POINT ( 'NONE',  ( 39.31379013062058192, -274.5187136260051943, -274.0428914934993827 ) ) ;
#17888=CARTESIAN_POINT ( 'NONE',  ( -94.68934645725113342, -271.2205475670941723, -222.0067555394310261 ) ) ;
#17889=CARTESIAN_POINT ( 'NONE',  ( -55.90940225614659909, -296.7119844954328869, -344.4816058991301020 ) ) ;
#17893=CARTESIAN_POINT ( 'NONE',  ( -105.8587019241274021, -285.9784302318867049, -244.2910865683883230 ) ) ;
#17894=CARTESIAN_POINT ( 'NONE',  ( 28.88980644139570231, -283.8031981469814582, -307.7157132501973820 ) ) ;
#17895=CARTESIAN_POINT ( 'NONE',  ( -104.2098807475242950, -283.5037726830101974, -299.8998906126874999 ) ) ;
#17896=CARTESIAN_POINT ( 'NONE',  ( -26.92855561026095756, -275.3174022520358903, -343.4227825891136376 ) ) ;
#17897=CARTESIAN_POINT ( 'NONE',  ( -38.88743911569032718, -284.9321276517055139, -344.5929297332987744 ) ) ;
#17898=CARTESIAN_POINT ( 'NONE',  ( -108.8495197728233705, -276.7985453130717701, -288.2272198505789902 ) ) ;
#17899=CARTESIAN_POINT ( 'NONE',  ( -31.32800131403647725, -275.2095288573261200, -197.2863761609956725 ) ) ;
#17901=CARTESIAN_POINT ( 'NONE',  ( -48.10629391742389771, -280.7214930502006496, -194.2266236132717268 ) ) ;
#17904=CARTESIAN_POINT ( 'NONE',  ( -43.58843769956197889, -287.8345778333856515, -194.8018668970822205 ) ) ;
#17905=CARTESIAN_POINT ( 'NONE',  ( -3.077160550970305053, -293.7843424804066217, -335.0027690669103890 ) ) ;
#17907=CARTESIAN_POINT ( 'NONE',  ( -112.5385412501642719, -290.1029234668242225, -254.2133834058313369 ) ) ;
#17908=CARTESIAN_POINT ( 'NONE',  ( -7.830588247316364381, -284.6841226726079412, -202.4857300217522891 ) ) ;
#17909=CARTESIAN_POINT ( 'NONE',  ( 26.89048318388064729, -285.6383751426846516, -234.3457915549133759 ) ) ;
#17910=CARTESIAN_POINT ( 'NONE',  ( -77.79046375480390907, -289.7405051465075871, -208.3782854139334972 ) ) ;
#17912=CARTESIAN_POINT ( 'NONE',  ( -110.7150508492322700, -285.7138046583366418, -273.6712645020565446 ) ) ;
#17913=CARTESIAN_POINT ( 'NONE',  ( -74.37149863358020241, -275.5444467015143459, -335.5822393489199840 ) ) ;
#17914=CARTESIAN_POINT ( 'NONE',  ( 36.72197811232332754, -286.1791198311559583, -288.3329846976881186 ) ) ;
#17915=CARTESIAN_POINT ( 'NONE',  ( -35.23073474381349257, -288.0787840962679525, -195.3780250453162637 ) ) ;
#17916=CARTESIAN_POINT ( 'NONE',  ( 37.86769054303137239, -285.5671982581714019, -271.5483714285646784 ) ) ;
#17918=CARTESIAN_POINT ( 'NONE',  ( -64.13031593051653090, -284.3516778530453166, -338.5210659848444834 ) ) ;
#17919=CARTESIAN_POINT ( 'NONE',  ( -51.31882272647337828, -291.2306304217091792, -344.2168453672753685 ) ) ;
#17921=CARTESIAN_POINT ( 'NONE',  ( -112.2221283039967261, -298.3385691411418748, -280.8545720266008061 ) ) ;
#17922=CARTESIAN_POINT ( 'NONE',  ( 19.49643042900759937, -278.8735348455500684, -221.4085070258459496 ) ) ;
#17923=CARTESIAN_POINT ( 'NONE',  ( 27.92062554659392148, -292.2165256299355747, -229.7021124312570635 ) ) ;
#17924=CARTESIAN_POINT ( 'NONE',  ( -88.66764493470971331, -295.7175498362159374, -217.2606677287537025 ) ) ;
#17925=CARTESIAN_POINT ( 'NONE',  ( 36.19605775320617624, -280.2497566681219610, -271.3369076827034974 ) ) ;
#17926=CARTESIAN_POINT ( 'NONE',  ( -54.52057962059964069, -271.9095451280041402, -197.9304594582519599 ) ) ;
#17927=CARTESIAN_POINT ( 'NONE',  ( -15.42993453999099351, -296.0778288366647075, -340.5653331691756307 ) ) ;
#17928=CARTESIAN_POINT ( 'NONE',  ( 82.61707336526248469, -302.0539871969763226, -195.3101965168185075 ) ) ;
#17929=CARTESIAN_POINT ( 'NONE',  ( -30.54182987992833631, -296.6157088357578573, -194.0561673880331455 ) ) ;
#17930=CARTESIAN_POINT ( 'NONE',  ( 16.82328374188123377, -292.5341632022899603, -323.7287901156560110 ) ) ;
#17931=CARTESIAN_POINT ( 'NONE',  ( -64.30426354947856282, -293.1185809685653680, -201.8756179379270463 ) ) ;
#17933=CARTESIAN_POINT ( 'NONE',  ( 2.319469534305223846, -293.4009671579829046, -208.8227126230175656 ) ) ;
#17935=CARTESIAN_POINT ( 'NONE',  ( -49.84594460838042806, -281.2308681745444119, -344.7243461393659913 ) ) ;
#17936=CARTESIAN_POINT ( 'NONE',  ( -23.51883577991246099, -294.8706522354275421, -342.0920666986595506 ) ) ;
#17937=CARTESIAN_POINT ( 'NONE',  ( -35.89919520043400070, -283.0345628644328713, -347.3607219302351155 ) ) ;
#17938=CARTESIAN_POINT ( 'NONE',  ( 16.18541838600518901, -282.7241604108434103, -216.9570936029969914 ) ) ;
#17939=CARTESIAN_POINT ( 'NONE',  ( -112.9766573518263471, -284.4014519225808044, -255.7626271358629992 ) ) ;
#17940=CARTESIAN_POINT ( 'NONE',  ( -111.2333342016190585, -288.3986596520966827, -282.2763623087900555 ) ) ;
#17942=CARTESIAN_POINT ( 'NONE',  ( 38.83566919842929366, -280.0985560234222476, -275.6324650527377003 ) ) ;
#17943=CARTESIAN_POINT ( 'NONE',  ( 37.80264758640984724, -286.6649037824816446, -285.6849398751988929 ) ) ;
#17944=DIRECTION ( 'NONE',  ( 0.9951408606192332362, 1.205805641958552022E-17, 0.09846150276129254919 ) ) ;
#17945=CARTESIAN_POINT ( 'NONE',  ( 2.013500102684104398, -296.1163451210549056, -332.8524822916819517 ) ) ;
#17946=CARTESIAN_POINT ( 'NONE',  ( 5.555600154180043049, -277.9087550779553908, -333.5942415821975260 ) ) ;
#17947=CARTESIAN_POINT ( 'NONE',  ( -19.52528915047310676, -279.9542605156218542, -199.4945267803107640 ) ) ;
#17948=CARTESIAN_POINT ( 'NONE',  ( 37.08203665545636341, -293.4709804389500505, -250.5591165819264745 ) ) ;
#17949=CARTESIAN_POINT ( 'NONE',  ( -102.7808759551754036, -283.1336685982954577, -232.4810949917221023 ) ) ;
#17950=CARTESIAN_POINT ( 'NONE',  ( -96.33944084527684026, -279.9167293191851513, -316.6673512941497393 ) ) ;
#17951=CARTESIAN_POINT ( 'NONE',  ( 4.648329915294786119, -291.6929981418353464, -210.2968972892569184 ) ) ;
#17952=CARTESIAN_POINT ( 'NONE',  ( -102.6243353615422222, -271.0489455335326738, -232.9980859303907437 ) ) ;
#17955=CARTESIAN_POINT ( 'NONE',  ( 35.48527500345447550, -293.1369055841996669, -276.2109158189680329 ) ) ;
#17957=CARTESIAN_POINT ( 'NONE',  ( 30.91033621190086578, -284.8380690714489560, -254.8156830097664738 ) ) ;
#17958=CARTESIAN_POINT ( 'NONE',  ( -114.0191301341673835, -271.8211713909706191, -264.6280860948100440 ) ) ;
#17959=CARTESIAN_POINT ( 'NONE',  ( 7.242866786761873676, -287.9604952569976604, -208.1226151188525648 ) ) ;
#17960=CARTESIAN_POINT ( 'NONE',  ( -58.69115764644078581, -289.1692586464731107, -340.2222362731490648 ) ) ;
#17961=CARTESIAN_POINT ( 'NONE',  ( -74.34482963965119495, -279.0739464559936209, -334.0908297273024914 ) ) ;
#17962=CARTESIAN_POINT ( 'NONE',  ( -99.97003332532584352, -274.6852543939538691, -231.3209810034608438 ) ) ;
#17963=CARTESIAN_POINT ( 'NONE',  ( 2.934630619526648498, -279.4006366701439674, -208.9409556386853524 ) ) ;
#17965=CARTESIAN_POINT ( 'NONE',  ( -97.32720108050966701, -296.8656143773355325, -222.1171135140552053 ) ) ;
#17966=CARTESIAN_POINT ( 'NONE',  ( -111.2156214725146839, -292.3537753134795594, -279.5239746591864218 ) ) ;
#17967=CARTESIAN_POINT ( 'NONE',  ( 25.81826575643291477, -294.5835893717372187, -227.6390108249181594 ) ) ;
#17970=CARTESIAN_POINT ( 'NONE',  ( -96.63644385673210024, -290.6064540176594164, -313.1165390954720351 ) ) ;
#17972=CARTESIAN_POINT ( 'NONE',  ( 34.29264416751010458, -291.3738325663738920, -245.5277576387058218 ) ) ;
#17974=CARTESIAN_POINT ( 'NONE',  ( -65.53821522606727967, -298.0268086569568595, -198.6752323913819396 ) ) ;
#17975=CARTESIAN_POINT ( 'NONE',  ( -109.6427289972625658, -272.2029407733185735, -259.5013167817942303 ) ) ;
#17977=LINE ( 'NONE', #24607, #76400 ) ;
#17978=CARTESIAN_POINT ( 'NONE',  ( -94.92228125629038971, -291.3892706161867636, -320.4329107491910804 ) ) ;
#17979=CARTESIAN_POINT ( 'NONE',  ( -115.3288506153726871, -298.8376638359844719, -288.1938231032136741 ) ) ;
#17980=CARTESIAN_POINT ( 'NONE',  ( -95.56410301845868105, -287.2010402643243197, -223.3282454972648168 ) ) ;
#17981=CARTESIAN_POINT ( 'NONE',  ( -31.16358464767422731, -272.1301938694913360, -195.7702764445280934 ) ) ;
#17982=CARTESIAN_POINT ( 'NONE',  ( 10.39005413820319923, -276.6366541941227410, -213.1710137120338970 ) ) ;
#17983=CARTESIAN_POINT ( 'NONE',  ( -0.5235883853854483849, -290.6252841494993504, -205.6490530696761141 ) ) ;
#17984=CARTESIAN_POINT ( 'NONE',  ( -56.58702471676015477, -279.1579247533197758, -343.6950406279113963 ) ) ;
#17986=CARTESIAN_POINT ( 'NONE',  ( 21.08638295824463782, -281.5170183977454030, -314.3141549924685592 ) ) ;
#17987=CARTESIAN_POINT ( 'NONE',  ( -67.57404601996459803, -278.5192752884484548, -340.8415959338715879 ) ) ;
#17988=CARTESIAN_POINT ( 'NONE',  ( 37.47438529173152233, -280.5546241949439263, -286.8704121074773639 ) ) ;
#17989=CARTESIAN_POINT ( 'NONE',  ( -57.01831460352683223, -168.7166579112505076, -361.2910810254234093 ) ) ;
#17990=CARTESIAN_POINT ( 'NONE',  ( 39.39533236147819650, -276.4675469492279944, -268.3000364723632174 ) ) ;
#17992=CARTESIAN_POINT ( 'NONE',  ( -89.70131972699893197, -274.8501301295296457, -214.7805831402981482 ) ) ;
#17994=CARTESIAN_POINT ( 'NONE',  ( 10.64812456238590066, -296.9090924074130271, -330.4860931364851808 ) ) ;
#17998=CARTESIAN_POINT ( 'NONE',  ( -76.02020901471033199, -290.6618753314619994, -332.6363058482935458 ) ) ;
#17999=CARTESIAN_POINT ( 'NONE',  ( 38.34021232037498095, -289.3984532023920337, -277.1598046428026692 ) ) ;
#18000=CARTESIAN_POINT ( 'NONE',  ( -107.0518137728636816, -289.6073988583702885, -292.5375279606629420 ) ) ;
#18001=CARTESIAN_POINT ( 'NONE',  ( -4.794276594578900763, -285.9770882108968522, -200.6460398081742937 ) ) ;
#18003=CARTESIAN_POINT ( 'NONE',  ( 36.50304705240625935, -279.9648481492842507, -271.3445336252290190 ) ) ;
#18004=CARTESIAN_POINT ( 'NONE',  ( 22.97897273797579487, -290.0073499000262700, -313.6309909518141126 ) ) ;
#18005=CARTESIAN_POINT ( 'NONE',  ( -61.78276150045344650, -281.8553734777087243, -339.9371088017694547 ) ) ;
#18006=CARTESIAN_POINT ( 'NONE',  ( -69.97424247316737933, -280.9282175235711634, -204.4961280445561442 ) ) ;
#18007=CARTESIAN_POINT ( 'NONE',  ( 38.85852485267836443, -288.6153405054805035, -280.0814623336628983 ) ) ;
#18008=CARTESIAN_POINT ( 'NONE',  ( -104.3253024600627441, -278.6510317413237772, -299.6629466611464636 ) ) ;
#18009=CARTESIAN_POINT ( 'NONE',  ( -110.8468058300933308, -289.6189627239074298, -248.7970702489311918 ) ) ;
#18010=CARTESIAN_POINT ( 'NONE',  ( -105.6359288366484606, -284.8988409717413219, -305.6916251268866063 ) ) ;
#18011=CARTESIAN_POINT ( 'NONE',  ( -60.49737871820320834, -286.2521588366652168, -196.9343270369304264 ) ) ;
#18012=CARTESIAN_POINT ( 'NONE',  ( -88.89278703546426641, -283.9676730958867665, -322.1184815215181629 ) ) ;
#18015=CARTESIAN_POINT ( 'NONE',  ( -6.413199518535557253, -294.3144447141544333, -201.1825231115184920 ) ) ;
#18016=CARTESIAN_POINT ( 'NONE',  ( 39.00876406373024707, -292.3082015038104373, -276.0194636441065086 ) ) ;
#18017=CARTESIAN_POINT ( 'NONE',  ( 19.18809629456653809, -273.9531950305727150, -223.8015801276337129 ) ) ;
#18019=CARTESIAN_POINT ( 'NONE',  ( -94.58125694300041175, -295.2029220962525642, -321.7319407562005154 ) ) ;
#18020=CARTESIAN_POINT ( 'NONE',  ( -3.298921860933128336, -290.9901752331776947, -205.0021323581624983 ) ) ;
#18021=CARTESIAN_POINT ( 'NONE',  ( -61.36295055479155280, -293.6081528662633104, -340.4222530457843163 ) ) ;
#18022=CARTESIAN_POINT ( 'NONE',  ( -72.83233706808053398, -292.7763400831755121, -206.0580258984577142 ) ) ;
#18024=CARTESIAN_POINT ( 'NONE',  ( -2.873279564846140222, -290.5064174230686831, -203.5488127789022599 ) ) ;
#18025=CARTESIAN_POINT ( 'NONE',  ( 37.40978467044119071, -295.6383167608520353, -277.0590636709445675 ) ) ;
#18026=CARTESIAN_POINT ( 'NONE',  ( 14.25763484092335887, -289.2461596953247636, -322.3314660537604937 ) ) ;
#18027=CARTESIAN_POINT ( 'NONE',  ( -41.27287486526417837, -279.0812758069678239, -345.6266372181603401 ) ) ;
#18028=CARTESIAN_POINT ( 'NONE',  ( -98.49574850924500424, -276.7293206268953440, -316.5149732037925787 ) ) ;
#18029=CARTESIAN_POINT ( 'NONE',  ( 30.62114302869646210, -298.0799046342134488, -193.5315563099809992 ) ) ;
#18030=CARTESIAN_POINT ( 'NONE',  ( -21.45709149045410413, -275.0856687575517299, -342.7025081007390099 ) ) ;
#18031=CARTESIAN_POINT ( 'NONE',  ( -88.50290385550056271, -277.4083945310232480, -216.2173105567106575 ) ) ;
#18032=CARTESIAN_POINT ( 'NONE',  ( -74.95918653625092531, -275.9444142133216360, -336.6284940595022022 ) ) ;
#18033=ADVANCED_FACE ( 'NONE', ( #73941 ), #9056, .F. ) ;
#18034=CARTESIAN_POINT ( 'NONE',  ( -92.57227568588936606, -294.5495288714236040, -318.8464456849785051 ) ) ;
#18036=CARTESIAN_POINT ( 'NONE',  ( -49.99186470170865704, -298.6894284096910610, -198.3015935408572830 ) ) ;
#18039=CARTESIAN_POINT ( 'NONE',  ( -84.16285887031533264, -287.7119377562086129, -329.4716425059943958 ) ) ;
#18040=CARTESIAN_POINT ( 'NONE',  ( 15.44825792080862570, -274.6574826638428135, -219.8675067066500333 ) ) ;
#18041=CARTESIAN_POINT ( 'NONE',  ( 38.29018392685653538, -287.3714282203288235, -255.9105777054480484 ) ) ;
#18042=CARTESIAN_POINT ( 'NONE',  ( -105.1993608477266520, -274.9768893016398579, -238.0289930122082467 ) ) ;
#18043=CARTESIAN_POINT ( 'NONE',  ( -105.6195421794715941, -294.1480482802759298, -301.1173586129912110 ) ) ;
#18044=CARTESIAN_POINT ( 'NONE',  ( -99.66352008639135818, -283.1511254564550200, -315.3961251892413884 ) ) ;
#18046=CARTESIAN_POINT ( 'NONE',  ( -110.7826118108331741, -276.7481238899337654, -255.0860738245242487 ) ) ;
#18048=CARTESIAN_POINT ( 'NONE',  ( -110.6412360897021188, -289.4082884483579505, -265.6951657635079300 ) ) ;
#18051=CARTESIAN_POINT ( 'NONE',  ( -109.6741961782062020, -288.8069350171326732, -250.5366213644957725 ) ) ;
#18052=CARTESIAN_POINT ( 'NONE',  ( -29.93929056898641861, -275.6676698235258982, -197.0405063863528028 ) ) ;
#18053=CARTESIAN_POINT ( 'NONE',  ( 38.59506268172602006, -282.8644978374809966, -261.4008997495978406 ) ) ;
#18054=CARTESIAN_POINT ( 'NONE',  ( 73.39505216521877173, -297.4518555997764793, -195.0430490344880639 ) ) ;
#18055=CARTESIAN_POINT ( 'NONE',  ( -76.12712328346938762, -283.5858777957122356, -332.2649855398151431 ) ) ;
#18056=CARTESIAN_POINT ( 'NONE',  ( -76.89610879619954176, -274.9361968461952301, -208.3061127740946858 ) ) ;
#18057=CARTESIAN_POINT ( 'NONE',  ( 33.66343321265914312, -276.1228331557512661, -252.7295336312109839 ) ) ;
#18058=CARTESIAN_POINT ( 'NONE',  ( 10.24384159414530693, -284.3963923786469081, -328.3991689218567558 ) ) ;
#18059=CARTESIAN_POINT ( 'NONE',  ( -85.50292996027178560, -272.2882151667443509, -215.0239310549584388 ) ) ;
#18062=CARTESIAN_POINT ( 'NONE',  ( 22.28528703165126856, -294.0396495093075941, -319.1016519084193988 ) ) ;
#18063=CARTESIAN_POINT ( 'NONE',  ( -100.4074896745002121, -285.9912218275712235, -310.3896868822066040 ) ) ;
#18065=CARTESIAN_POINT ( 'NONE',  ( -111.2586520408596868, -276.4809262143062369, -234.7283546768995564 ) ) ;
#18066=CARTESIAN_POINT ( 'NONE',  ( -114.0713048191169463, -277.6980648889752388, -274.4509326489190926 ) ) ;
#18067=CARTESIAN_POINT ( 'NONE',  ( -71.56561616223670796, -287.8965877215275668, -338.4431566515374925 ) ) ;
#18068=CARTESIAN_POINT ( 'NONE',  ( -64.29106800550495393, -284.9304544015237184, -338.9500334413642122 ) ) ;
#18069=CARTESIAN_POINT ( 'NONE',  ( -83.62318655960478964, -279.4568709248052869, -328.1851628299783101 ) ) ;
#18070=CARTESIAN_POINT ( 'NONE',  ( 9.435613885606153772, -288.1064320772111387, -209.9418397267265846 ) ) ;
#18071=CARTESIAN_POINT ( 'NONE',  ( -13.70199456395707571, -282.3590026441876262, -199.1292238622698676 ) ) ;
#18072=CARTESIAN_POINT ( 'NONE',  ( 26.14336544449704647, -275.1435071581625493, -226.7642883875858502 ) ) ;
#18073=CARTESIAN_POINT ( 'NONE',  ( -114.0793033075686793, -278.2983300078909679, -277.3289659113175958 ) ) ;
#18074=CARTESIAN_POINT ( 'NONE',  ( -111.6511860468581290, -298.5293127653650345, -265.9549293871266400 ) ) ;
#18076=CARTESIAN_POINT ( 'NONE',  ( 10.59707575819634329, -277.1948066931274184, -210.1954327657594490 ) ) ;
#18077=CARTESIAN_POINT ( 'NONE',  ( 18.28230932294182765, -296.8810154162835602, -194.6137105603779673 ) ) ;
#18078=CARTESIAN_POINT ( 'NONE',  ( -21.64590741762824067, -276.3532587977351795, -341.7688153884450912 ) ) ;
#18079=CARTESIAN_POINT ( 'NONE',  ( -15.90327380157685866, -275.5283849561884040, -196.7642256439629875 ) ) ;
#18080=CARTESIAN_POINT ( 'NONE',  ( -30.45906869755862800, -287.9003832277448396, -196.6169872058072201 ) ) ;
#18081=CARTESIAN_POINT ( 'NONE',  ( -113.4311038434072714, -298.1532039758272958, -263.9481717307529607 ) ) ;
#18082=CARTESIAN_POINT ( 'NONE',  ( -65.44347433371051181, -296.6165405443485383, -341.6374502665573800 ) ) ;
#18083=CARTESIAN_POINT ( 'NONE',  ( 18.07920354488868497, -294.8486975101263283, -220.0004401667031289 ) ) ;
#18084=CARTESIAN_POINT ( 'NONE',  ( -66.76772219179306944, -277.6655957177939058, -201.5420688903798521 ) ) ;
#18085=CARTESIAN_POINT ( 'NONE',  ( -1.289670350696733969, -282.4544997042830801, -205.2338168861113274 ) ) ;
#18086=CARTESIAN_POINT ( 'NONE',  ( -91.06857115018763693, -295.3619118662326741, -218.7632322667241453 ) ) ;
#18087=CARTESIAN_POINT ( 'NONE',  ( -63.46355892975361002, -285.2493971380450262, -341.4804119374946367 ) ) ;
#18088=CARTESIAN_POINT ( 'NONE',  ( -5.652630567788729188, -285.3992527417561291, -204.2410801963400218 ) ) ;
#18089=CARTESIAN_POINT ( 'NONE',  ( -105.6297312391304359, -263.1519871882180723, -317.3200005741121004 ) ) ;
#18091=CARTESIAN_POINT ( 'NONE',  ( 18.68071328570327694, -286.5540901638994455, -223.5060017140951913 ) ) ;
#18092=EDGE_LOOP ( 'NONE', ( #54036, #2952, #91460, #50386 ) ) ;
#18093=CARTESIAN_POINT ( 'NONE',  ( -113.5950452014927379, -285.5291007883886891, -278.5415748413252572 ) ) ;
#18094=CARTESIAN_POINT ( 'NONE',  ( 35.37545181723947252, -275.9732145410503676, -277.0171903743586199 ) ) ;
#18095=CARTESIAN_POINT ( 'NONE',  ( 38.58375897387485765, -286.2192895141771487, -260.1958153054453646 ) ) ;
#18096=CARTESIAN_POINT ( 'NONE',  ( -101.4180963075515507, -290.0297646582602056, -228.1266961355314891 ) ) ;
#18097=CARTESIAN_POINT ( 'NONE',  ( 35.10164134661182089, -282.1703452812040496, -244.8098595320705613 ) ) ;
#18099=CARTESIAN_POINT ( 'NONE',  ( -74.68567290369099965, -281.0845501752829705, -203.8168811883388685 ) ) ;
#18100=CARTESIAN_POINT ( 'NONE',  ( 22.85612142997651119, -281.2426715117946969, -222.3613495282661745 ) ) ;
#18102=CARTESIAN_POINT ( 'NONE',  ( -67.74223827176246004, -286.9809262143061233, -333.4151289067050357 ) ) ;
#18103=CARTESIAN_POINT ( 'NONE',  ( -83.59145992945265391, -219.8537403536915349, -352.6472634170126526 ) ) ;
#18105=CARTESIAN_POINT ( 'NONE',  ( 32.99342612457994761, -277.8861982004544871, -296.0656774936185229 ) ) ;
#18106=CARTESIAN_POINT ( 'NONE',  ( 4.790628490442398579, -57.97448044145017576, -354.2496948606743103 ) ) ;
#18108=CARTESIAN_POINT ( 'NONE',  ( 26.96347060040966781, -280.0826325642604502, -308.3669161624852109 ) ) ;
#18109=CARTESIAN_POINT ( 'NONE',  ( -16.75952356001461752, -296.5501350731234993, -343.5617022503755038 ) ) ;
#18110=CARTESIAN_POINT ( 'NONE',  ( -102.8631988861991289, -295.4605631668603110, -302.8919788410278215 ) ) ;
#18111=CARTESIAN_POINT ( 'NONE',  ( -101.6290880532886405, -290.6169941463634245, -227.9966399342466161 ) ) ;
#18113=CARTESIAN_POINT ( 'NONE',  ( -112.8047378861226093, -295.2791273407638641, -258.2810093332199699 ) ) ;
#18114=CARTESIAN_POINT ( 'NONE',  ( 33.84824440399329148, -286.2084714786589643, -290.0038920776575537 ) ) ;
#18115=CARTESIAN_POINT ( 'NONE',  ( 35.92933724591973288, -295.2568409881761795, -258.3561569091314709 ) ) ;
#18116=CARTESIAN_POINT ( 'NONE',  ( -4.388352754425544511, -287.8110998014808501, -204.6700198311277745 ) ) ;
#18118=CARTESIAN_POINT ( 'NONE',  ( 24.70319955045539473, -295.0954095058709754, -315.5855944460318483 ) ) ;
#18119=CARTESIAN_POINT ( 'NONE',  ( -110.0563141808517003, -285.1448226521748097, -262.7498669716907784 ) ) ;
#18120=CARTESIAN_POINT ( 'NONE',  ( -111.9227573999169607, -295.1265798582989532, -287.9014542500962648 ) ) ;
#18121=CARTESIAN_POINT ( 'NONE',  ( -102.1595363065640498, -290.8118206242222072, -311.7240932340248492 ) ) ;
#18122=CARTESIAN_POINT ( 'NONE',  ( -112.5811137997226865, -291.2464985321876156, -254.2192117478826390 ) ) ;
#18123=CARTESIAN_POINT ( 'NONE',  ( -107.7252383329497576, -290.4606925366467181, -289.9163623409639854 ) ) ;
#18126=CARTESIAN_POINT ( 'NONE',  ( -86.67621203822126574, -299.2356916232678827, -212.7905346530961879 ) ) ;
#18127=CARTESIAN_POINT ( 'NONE',  ( -83.32939574910948011, -272.2329275806613964, -209.0318582419886297 ) ) ;
#18128=CARTESIAN_POINT ( 'NONE',  ( -16.07558768771819047, -281.8290384852472243, -340.4407934189530351 ) ) ;
#18129=CARTESIAN_POINT ( 'NONE',  ( 25.28046480523453710, -274.4669971186978614, -225.6396809806910255 ) ) ;
#18130=CARTESIAN_POINT ( 'NONE',  ( -108.2753891595561839, -294.7704246917772934, -290.3390937019854050 ) ) ;
#18131=CARTESIAN_POINT ( 'NONE',  ( -69.76995504129746450, -279.3441004804227532, -337.1529813944812872 ) ) ;
#18132=CARTESIAN_POINT ( 'NONE',  ( -32.58867434441228284, -272.2522469987749787, -196.2654923021844979 ) ) ;
#18133=CARTESIAN_POINT ( 'NONE',  ( -40.55060778842110381, -299.2160173004481294, -197.0216068422801925 ) ) ;
#18134=CARTESIAN_POINT ( 'NONE',  ( -69.40509320019954487, -298.6996137152854089, -204.4356684245572922 ) ) ;
#18136=CARTESIAN_POINT ( 'NONE',  ( -84.73494010419553035, -299.0113074292253259, -210.6926906699645770 ) ) ;
#18137=CARTESIAN_POINT ( 'NONE',  ( -105.3477705462717040, -270.9974771543297152, -237.9022026277494604 ) ) ;
#18138=CARTESIAN_POINT ( 'NONE',  ( 12.43034001889411222, -294.9884195360733656, -323.9714860499759084 ) ) ;
#18139=CARTESIAN_POINT ( 'NONE',  ( 2.575236969764949091, -291.1732212437169665, -208.4783142036073684 ) ) ;
#18141=CARTESIAN_POINT ( 'NONE',  ( -7.720073655555841796, -274.9223180753100451, -199.2969198332054361 ) ) ;
#18142=CARTESIAN_POINT ( 'NONE',  ( -37.82691618514939336, -298.3791909823559081, -197.3415859910845711 ) ) ;
#18143=CARTESIAN_POINT ( 'NONE',  ( 16.66543480844003255, -284.2688982524047105, -322.9869758288136836 ) ) ;
#18144=CARTESIAN_POINT ( 'NONE',  ( -30.27720841372053684, -281.6493745725233566, -346.5411102987293930 ) ) ;
#18145=CARTESIAN_POINT ( 'NONE',  ( -56.90611539612606862, -276.6464998373929802, -344.7837432606136758 ) ) ;
#18147=CARTESIAN_POINT ( 'NONE',  ( -80.73010197126023968, -282.8547259652038406, -329.3312706299911383 ) ) ;
#18148=CARTESIAN_POINT ( 'NONE',  ( -41.49395986215245102, -281.1040366486934658, -345.4640943208969475 ) ) ;
#18150=CARTESIAN_POINT ( 'NONE',  ( 14.13060180820468936, -274.8870813091570540, -323.0246247685816456 ) ) ;
#18151=CARTESIAN_POINT ( 'NONE',  ( -64.59782538862290835, -281.6966279207716184, -200.4342570663369827 ) ) ;
#18154=CARTESIAN_POINT ( 'NONE',  ( -80.77747054860677167, -271.8738210070736159, -207.6890882135760421 ) ) ;
#18155=CARTESIAN_POINT ( 'NONE',  ( -111.2580287891604485, -280.3764921234789540, -284.0847209193519234 ) ) ;
#18157=CARTESIAN_POINT ( 'NONE',  ( -90.89986402906950502, -287.2193120737205732, -217.0616125765146478 ) ) ;
#18160=CARTESIAN_POINT ( 'NONE',  ( 36.84248808864709446, -285.4059526134255407, -258.9873166894478231 ) ) ;
#18162=CARTESIAN_POINT ( 'NONE',  ( -110.1279612694756338, -295.4760791475494557, -260.5284142102742067 ) ) ;
#18163=CARTESIAN_POINT ( 'NONE',  ( -105.1860589060041207, -288.2913466964842542, -300.6213360324474024 ) ) ;
#18164=CARTESIAN_POINT ( 'NONE',  ( 64.33209501061345748, 48.33985520751024723, -319.1928417150128325 ) ) ;
#18165=CARTESIAN_POINT ( 'NONE',  ( -97.69499511117089696, -295.1596666381653336, -225.8143914365068383 ) ) ;
#18166=CARTESIAN_POINT ( 'NONE',  ( -30.92270915973745815, -284.6117327519158948, -194.3117388756587616 ) ) ;
#18167=CARTESIAN_POINT ( 'NONE',  ( 22.47216124325061415, -283.7506862935746881, -313.6117163196296360 ) ) ;
#18168=CARTESIAN_POINT ( 'NONE',  ( -64.90578011014414983, -281.6471356910333839, -341.1861210966881686 ) ) ;
#18169=CARTESIAN_POINT ( 'NONE',  ( -61.25501244800953060, -289.3715228502236414, -339.3332391177663112 ) ) ;
#18170=CARTESIAN_POINT ( 'NONE',  ( -43.82091183182579641, -281.3940838636777357, -197.0070357235220513 ) ) ;
#18171=CARTESIAN_POINT ( 'NONE',  ( -37.01785133431243935, -280.8591444631121021, -197.2003576699578673 ) ) ;
#18172=CARTESIAN_POINT ( 'NONE',  ( 34.81779940107080762, -289.8110128755184292, -292.1180423218158353 ) ) ;
#18174=CARTESIAN_POINT ( 'NONE',  ( -113.7750372036288411, -296.8354465289459654, -261.0366883487457130 ) ) ;
#18176=CARTESIAN_POINT ( 'NONE',  ( -24.15960795104886927, -274.2158917917183771, -194.4437033385387963 ) ) ;
#18178=CARTESIAN_POINT ( 'NONE',  ( -107.5717539381432175, -292.2026357477438978, -295.6511623316070541 ) ) ;
#18180=CARTESIAN_POINT ( 'NONE',  ( -4.829096099716510437, -276.9805209788416391, -202.7746430608542312 ) ) ;
#18182=CARTESIAN_POINT ( 'NONE',  ( 17.54664569466083179, -274.2695623513662895, -321.7157469823216616 ) ) ;
#18184=CARTESIAN_POINT ( 'NONE',  ( -3.601533979201898106, -293.0142652762226589, -338.6986365584622263 ) ) ;
#18185=CARTESIAN_POINT ( 'NONE',  ( -27.26793590769204556, -273.5320073009398811, -197.9056457494495191 ) ) ;
#18186=CARTESIAN_POINT ( 'NONE',  ( -109.0203320172620494, -291.8486196019856038, -287.4748985430444463 ) ) ;
#18187=CARTESIAN_POINT ( 'NONE',  ( 20.99330678552420437, -283.9455359496082565, -315.9132966880353592 ) ) ;
#18188=CARTESIAN_POINT ( 'NONE',  ( -56.06213042052504392, -293.2410307243430907, -196.2245256439732373 ) ) ;
#18189=CARTESIAN_POINT ( 'NONE',  ( -4.829022191148051313, -293.7866085262849083, -201.1063416257239282 ) ) ;
#18190=CARTESIAN_POINT ( 'NONE',  ( -15.59485231117861481, -294.5962133917923893, -340.0998296046340101 ) ) ;
#18191=CARTESIAN_POINT ( 'NONE',  ( 23.60131616392930809, -290.1470718771006432, -314.0755253990889173 ) ) ;
#18192=CARTESIAN_POINT ( 'NONE',  ( -1.632255045848221009, -282.7587562147315907, -338.5801441881794176 ) ) ;
#18193=CARTESIAN_POINT ( 'NONE',  ( -100.3354151751951377, -295.1916321699050059, -228.6110057608879629 ) ) ;
#18194=CARTESIAN_POINT ( 'NONE',  ( -90.43967588808307312, -283.6121212476750770, -326.1980611174371916 ) ) ;
#18195=CARTESIAN_POINT ( 'NONE',  ( 34.43478431926597239, -277.2648973475054959, -249.6831612301122902 ) ) ;
#18196=CARTESIAN_POINT ( 'NONE',  ( -21.39648532958013050, -294.7662352645559736, -200.3538533559491555 ) ) ;
#18197=CARTESIAN_POINT ( 'NONE',  ( -107.5213509424310985, -276.3232438051216491, -298.9114610597084152 ) ) ;
#18199=CARTESIAN_POINT ( 'NONE',  ( -21.38087224186254076, -282.3496806299198738, -341.7100209162651936 ) ) ;
#18200=CARTESIAN_POINT ( 'NONE',  ( -79.70404211110033543, -280.6987563318910475, -206.4739675803249099 ) ) ;
#18201=CARTESIAN_POINT ( 'NONE',  ( 37.79568156391006539, -286.4128727583988621, -254.5750176337077164 ) ) ;
#18202=CARTESIAN_POINT ( 'NONE',  ( 7.269428477275335254, -294.4298706296019645, -211.3033393625548797 ) ) ;
#18203=CARTESIAN_POINT ( 'NONE',  ( 4.407634550606300827, -276.2048717232679564, -206.5534572840067824 ) ) ;
#18205=CARTESIAN_POINT ( 'NONE',  ( 36.10765709695770909, -276.5949543200039216, -248.7637435899196419 ) ) ;
#18206=CARTESIAN_POINT ( 'NONE',  ( -41.85870550146714208, -276.9439378589466969, -343.2338315069463874 ) ) ;
#18208=CARTESIAN_POINT ( 'NONE',  ( -99.22052059591496231, -275.1005702501601036, -228.5213059457727525 ) ) ;
#18209=CARTESIAN_POINT ( 'NONE',  ( -60.52295502680039618, -283.7506191254590817, -199.2087614083980043 ) ) ;
#18210=CARTESIAN_POINT ( 'NONE',  ( -50.55855099160432786, -291.5544947063978611, -194.5253800703103764 ) ) ;
#18211=CARTESIAN_POINT ( 'NONE',  ( -88.93470132794379879, -291.3630481201342377, -326.4378746738435666 ) ) ;
#18212=CARTESIAN_POINT ( 'NONE',  ( -19.98570428150715372, -291.2006857172567607, -199.0836611186962841 ) ) ;
#18214=CARTESIAN_POINT ( 'NONE',  ( -25.09783649236970504, -290.7800888239664800, -194.9376859815413070 ) ) ;
#18215=CARTESIAN_POINT ( 'NONE',  ( 28.75946473516069801, -292.7984424068595217, -239.2139817779631414 ) ) ;
#18217=CARTESIAN_POINT ( 'NONE',  ( -23.35476190864703838, -289.9571510257961222, -345.8196457278615981 ) ) ;
#18218=CARTESIAN_POINT ( 'NONE',  ( -91.37775038224786783, -279.9085582765397362, -221.1270043901050428 ) ) ;
#18219=CARTESIAN_POINT ( 'NONE',  ( -114.0573774903131579, -295.4462826281028356, -272.4476079983765544 ) ) ;
#18220=CARTESIAN_POINT ( 'NONE',  ( -85.45559725608460155, -286.0580012751763661, -210.3747387834109190 ) ) ;
#18221=CARTESIAN_POINT ( 'NONE',  ( -10.00544028538734231, -286.7326382377291338, -198.3427249654797890 ) ) ;
#18222=CARTESIAN_POINT ( 'NONE',  ( -86.94008692393909143, -284.0984581363721304, -324.0221513108425029 ) ) ;
#18223=CARTESIAN_POINT ( 'NONE',  ( 197.2159948018767750, 285.3705696945321506, -111.7930995898936430 ) ) ;
#18224=CARTESIAN_POINT ( 'NONE',  ( -96.30717022866939203, -238.7289040402379499, -340.4382983491259438 ) ) ;
#18225=CARTESIAN_POINT ( 'NONE',  ( -111.6101193260526685, -270.5214411657722167, -283.6473540868328769 ) ) ;
#18226=CARTESIAN_POINT ( 'NONE',  ( -6.217195794883286553, -275.8295935994290744, -336.5856925556955161 ) ) ;
#18227=CARTESIAN_POINT ( 'NONE',  ( 20.25682744417047587, -275.1097319319255234, -315.7314752650584637 ) ) ;
#18228=CARTESIAN_POINT ( 'NONE',  ( -109.7908048430232242, -296.3869687276562672, -244.4641272472954654 ) ) ;
#18229=CARTESIAN_POINT ( 'NONE',  ( 200.0284319754563001, 285.7751889741193736, -96.47188040663559150 ) ) ;
#18230=CARTESIAN_POINT ( 'NONE',  ( 17.74622032706428598, -273.5047082110119732, -217.1943800814364351 ) ) ;
#18231=CARTESIAN_POINT ( 'NONE',  ( -40.84503458390711472, -275.7677631804482985, -196.3803512175339847 ) ) ;
#18233=CARTESIAN_POINT ( 'NONE',  ( 75.94312787335357484, -300.3792304208613473, -193.5787399965042823 ) ) ;
#18234=CARTESIAN_POINT ( 'NONE',  ( -94.99525922198839112, -290.4125029528289019, -315.2595586687715468 ) ) ;
#18235=CARTESIAN_POINT ( 'NONE',  ( -111.4335959565501213, -297.0993993742635553, -290.7216138842616715 ) ) ;
#18236=CARTESIAN_POINT ( 'NONE',  ( -54.58747309104741419, -298.3286030556758419, -195.3803856710929097 ) ) ;
#18237=CARTESIAN_POINT ( 'NONE',  ( 25.79372730310853612, -294.2215857037617184, -307.0069609605939718 ) ) ;
#18239=CARTESIAN_POINT ( 'NONE',  ( 0.3503353407831176769, -278.4747251098199285, -335.9080661585416578 ) ) ;
#18240=CARTESIAN_POINT ( 'NONE',  ( 24.54597781270600265, -280.4518560126807643, -224.6507009806088604 ) ) ;
#18241=CARTESIAN_POINT ( 'NONE',  ( -95.45242961043835805, -278.8683382162713542, -314.9318658767951433 ) ) ;
#18242=CARTESIAN_POINT ( 'NONE',  ( -12.18029923166183082, -278.4894790951256027, -342.1162313434322186 ) ) ;
#18243=CARTESIAN_POINT ( 'NONE',  ( -91.17211685321684911, -273.7530349604699609, -220.9434598797185174 ) ) ;
#18244=CARTESIAN_POINT ( 'NONE',  ( -35.78185683332136335, -296.6467796405653985, -196.7722720066452382 ) ) ;
#18246=CARTESIAN_POINT ( 'NONE',  ( -95.61303273711043005, -279.3367341394397272, -226.3693346183222275 ) ) ;
#18247=CARTESIAN_POINT ( 'NONE',  ( 4.766106513950871815, -275.4077043515254672, -206.0244268040095506 ) ) ;
#18248=CARTESIAN_POINT ( 'NONE',  ( 14.25866750302365737, -287.0301880852786667, -326.9191781763510676 ) ) ;
#18249=CARTESIAN_POINT ( 'NONE',  ( 8.273239772838325123, -276.6764850652170367, -210.8272796759979713 ) ) ;
#18250=CARTESIAN_POINT ( 'NONE',  ( -73.63393023854700914, -288.7441994783907262, -333.9009569047717605 ) ) ;
#18251=CARTESIAN_POINT ( 'NONE',  ( -95.73371541225596104, -284.5774979902026871, -220.2444228675807381 ) ) ;
#18252=CARTESIAN_POINT ( 'NONE',  ( -3.173229676874998351, -280.8342943871166426, -336.0296350206020293 ) ) ;
#18253=CARTESIAN_POINT ( 'NONE',  ( 36.10908704477111542, -280.0678305426265524, -265.8492691944703097 ) ) ;
#18254=CARTESIAN_POINT ( 'NONE',  ( -71.82396726941632892, -283.6724948674674920, -204.3892493326195563 ) ) ;
#18255=CARTESIAN_POINT ( 'NONE',  ( -46.28686702164063860, -291.1656739007130454, -344.8769959924919135 ) ) ;
#18256=CARTESIAN_POINT ( 'NONE',  ( -74.72115548864442758, -280.7481394762687614, -207.1369850336287470 ) ) ;
#18258=CARTESIAN_POINT ( 'NONE',  ( 7.630768672711631062, -294.6656197601119516, -210.2756722165279655 ) ) ;
#18259=CARTESIAN_POINT ( 'NONE',  ( -76.94499345125609580, -277.7696563499561648, -205.4499775751690436 ) ) ;
#18260=CARTESIAN_POINT ( 'NONE',  ( -3.813334485546819419, -277.2489309625477745, -335.3206543557988084 ) ) ;
#18261=CARTESIAN_POINT ( 'NONE',  ( -102.8074662133553829, -286.0600908035551129, -307.4023939802898440 ) ) ;
#18263=CARTESIAN_POINT ( 'NONE',  ( -73.71231011845847547, -291.4511664098068309, -336.6064918894743414 ) ) ;
#18264=CARTESIAN_POINT ( 'NONE',  ( -7.396603977905934713, -285.6319899620386309, -199.5412390962606537 ) ) ;
#18265=CARTESIAN_POINT ( 'NONE',  ( -94.90220160730498833, -289.5979389577954635, -224.1541500511134188 ) ) ;
#18267=CARTESIAN_POINT ( 'NONE',  ( -21.56336194408209295, -275.5305643681177798, -342.1928954265484322 ) ) ;
#18268=CARTESIAN_POINT ( 'NONE',  ( -76.32655861281827470, -293.7185316948441596, -333.5957865230379298 ) ) ;
#18271=CARTESIAN_POINT ( 'NONE',  ( -113.6747595037471825, -289.0573677027789472, -268.3534615565037598 ) ) ;
#18272=CARTESIAN_POINT ( 'NONE',  ( -60.24605010984494413, -287.3503279879221850, -200.2053543853141946 ) ) ;
#18273=CARTESIAN_POINT ( 'NONE',  ( -41.72480855978398750, -287.3464898732314055, -346.2343162145714928 ) ) ;
#18274=CARTESIAN_POINT ( 'NONE',  ( -30.49438800603590494, -287.5655683001523926, -197.0399350469283490 ) ) ;
#18276=CARTESIAN_POINT ( 'NONE',  ( -6.958753548722762972, -287.2641888718219434, -203.7930360852606668 ) ) ;
#18277=CARTESIAN_POINT ( 'NONE',  ( -11.73637659663021005, -294.3636547049829915, -199.4347522718885841 ) ) ;
#18278=CARTESIAN_POINT ( 'NONE',  ( -72.19855777007330744, -275.5893553945859935, -337.4151912561971471 ) ) ;
#18279=CARTESIAN_POINT ( 'NONE',  ( -82.53044031078729859, -277.9841851222492437, -332.6806338033837847 ) ) ;
#18280=CARTESIAN_POINT ( 'NONE',  ( -70.24808225174567156, -289.7017472216109013, -202.3428541240881202 ) ) ;
#18281=CARTESIAN_POINT ( 'NONE',  ( -113.0656290635832306, -278.3766548836172205, -284.3937385022919102 ) ) ;
#18282=CARTESIAN_POINT ( 'NONE',  ( -108.5816486204953861, -274.7547308092517255, -248.5930579052022154 ) ) ;
#18284=CARTESIAN_POINT ( 'NONE',  ( -112.3193019311769802, -282.5090842981202854, -273.7025136179500464 ) ) ;
#18286=CARTESIAN_POINT ( 'NONE',  ( -100.5064813694413601, -277.2217546671208765, -231.2621292671309732 ) ) ;
#18287=CARTESIAN_POINT ( 'NONE',  ( 33.70605846285116769, -279.8645509636867814, -294.5476827683453962 ) ) ;
#18289=CARTESIAN_POINT ( 'NONE',  ( -70.02181117564433066, -275.9546630496021180, -339.3298907177352248 ) ) ;
#18290=CARTESIAN_POINT ( 'NONE',  ( -106.4628282082076822, -298.4115358499530544, -244.6603995864948899 ) ) ;
#18291=CARTESIAN_POINT ( 'NONE',  ( 32.10660875633151790, -280.8921610010549443, -303.0196274746199379 ) ) ;
#18292=CARTESIAN_POINT ( 'NONE',  ( -110.4760157059144063, -297.4428570348641756, -274.2056377780733669 ) ) ;
#18293=CARTESIAN_POINT ( 'NONE',  ( -112.1220714190733503, -298.0714665907510721, -254.1383988901473288 ) ) ;
#18294=CARTESIAN_POINT ( 'NONE',  ( -63.31027542232896366, -273.3710172891319985, -202.1001258308832007 ) ) ;
#18295=CARTESIAN_POINT ( 'NONE',  ( 36.17193796058025157, -295.3615418253664870, -255.5036058404894277 ) ) ;
#18296=CARTESIAN_POINT ( 'NONE',  ( -0.9714313362855822032, -286.6880972751943091, -202.4921003638220043 ) ) ;
#18297=CARTESIAN_POINT ( 'NONE',  ( -2.064208747467626726, -274.7296795769385085, -337.4118755073128568 ) ) ;
#18298=CARTESIAN_POINT ( 'NONE',  ( -51.68738670159188331, -289.0641386776292734, -346.0129605326272895 ) ) ;
#18299=CARTESIAN_POINT ( 'NONE',  ( 35.78837939086074726, -286.5480692379236416, -265.5832576960827964 ) ) ;
#18300=CARTESIAN_POINT ( 'NONE',  ( -112.1902289058279649, -288.6131608084821778, -265.5968356571895015 ) ) ;
#18302=CARTESIAN_POINT ( 'NONE',  ( 138.4517698930976621, 181.0451598467585939, -241.7086681466011271 ) ) ;
#18303=CARTESIAN_POINT ( 'NONE',  ( 1.338852219042856007, -288.0277098621103278, -332.3434002230237638 ) ) ;
#18306=CARTESIAN_POINT ( 'NONE',  ( -100.8087374628426574, -286.0656555923040401, -227.0843837525586935 ) ) ;
#18307=CARTESIAN_POINT ( 'NONE',  ( 24.63160540069702620, -292.0076466708025578, -225.0606807299236891 ) ) ;
#18308=CARTESIAN_POINT ( 'NONE',  ( 38.08234982104021071, -283.2893557047473791, -281.2079195666263445 ) ) ;
#18309=EDGE_CURVE ( 'NONE', #32677, #20110, #62327, .T. ) ;
#18310=CARTESIAN_POINT ( 'NONE',  ( 37.76733636263002580, -282.6840814274303852, -255.8032709088620607 ) ) ;
#18311=CARTESIAN_POINT ( 'NONE',  ( -24.06757760856137551, -282.7111811987912802, -342.1441081391535022 ) ) ;
#18312=CARTESIAN_POINT ( 'NONE',  ( -13.11592327204001762, -278.7377274711695350, -341.3953809425485133 ) ) ;
#18313=CARTESIAN_POINT ( 'NONE',  ( -111.9686479433488557, -296.3141915376422162, -289.3832339960862896 ) ) ;
#18314=CARTESIAN_POINT ( 'NONE',  ( -74.53733417463298849, -274.8617465275469272, -206.9166063329775511 ) ) ;
#18315=CARTESIAN_POINT ( 'NONE',  ( -96.40063748384056908, -289.2008518132910808, -224.7114879200104554 ) ) ;
#18316=CARTESIAN_POINT ( 'NONE',  ( -77.67060023467416841, -296.4173304376658962, -209.0807987381998885 ) ) ;
#18318=CARTESIAN_POINT ( 'NONE',  ( 145.2857639756989272, -299.5541904835127980, -195.3611179825600175 ) ) ;
#18319=CARTESIAN_POINT ( 'NONE',  ( -91.77814820904001181, -285.7562145741270001, -321.1350022006735117 ) ) ;
#18320=CARTESIAN_POINT ( 'NONE',  ( 11.01410912075678006, -295.4807995822081352, -329.9544167945544473 ) ) ;
#18321=CARTESIAN_POINT ( 'NONE',  ( -110.3305589788174643, -285.2680457462315076, -265.4666329897965511 ) ) ;
#18322=CARTESIAN_POINT ( 'NONE',  ( -17.43051541249591807, -275.8600503434624329, -344.4985912031687576 ) ) ;
#18323=CARTESIAN_POINT ( 'NONE',  ( -94.64089820827537380, -291.9001253798788866, -219.0764742177589142 ) ) ;
#18324=CARTESIAN_POINT ( 'NONE',  ( -94.86300598963997288, -283.3686914473223624, -220.9711510432449586 ) ) ;
#18325=CARTESIAN_POINT ( 'NONE',  ( -42.05690816039972191, -292.3275221232314038, -193.5268085579447188 ) ) ;
#18326=CARTESIAN_POINT ( 'NONE',  ( -58.69125990973581963, -289.6691393703586641, -340.2443291341762688 ) ) ;
#18329=CARTESIAN_POINT ( 'NONE',  ( -93.40603346885242786, -239.0132304798418375, -338.5932674861245459 ) ) ;
#18330=CARTESIAN_POINT ( 'NONE',  ( -87.31066565302292304, -286.8907088013344833, -212.6213123086534154 ) ) ;
#18331=CARTESIAN_POINT ( 'NONE',  ( -37.37352853689063181, -274.5523547857346784, -350.3611179825600175 ) ) ;
#18332=CARTESIAN_POINT ( 'NONE',  ( 24.38331233821165966, -281.0184361849308630, -310.0049992628653968 ) ) ;
#18333=CARTESIAN_POINT ( 'NONE',  ( 18.88486615238925026, -275.9361726760148485, -322.9378955162528086 ) ) ;
#18334=CARTESIAN_POINT ( 'NONE',  ( -35.64617060351280742, -282.0736016005465672, -195.5342762581041711 ) ) ;
#18335=CARTESIAN_POINT ( 'NONE',  ( 201.0568784420084114, 286.4263594892526612, -96.83033023965205643 ) ) ;
#18337=CARTESIAN_POINT ( 'NONE',  ( -21.86321631561991197, -281.4322568384516217, -345.1877364426468375 ) ) ;
#18338=CARTESIAN_POINT ( 'NONE',  ( -111.7370907227955286, -282.4935987225156850, -276.4580564721121618 ) ) ;
#18339=CARTESIAN_POINT ( 'NONE',  ( 7.225731311262463485, -300.3629773498978466, -194.3612984979313296 ) ) ;
#18340=CARTESIAN_POINT ( 'NONE',  ( -73.32725876020806766, -296.0356526961273858, -333.9459275809488759 ) ) ;
#18342=CARTESIAN_POINT ( 'NONE',  ( 32.27353337005490630, -291.9241983709223405, -246.6449432311666499 ) ) ;
#18343=CARTESIAN_POINT ( 'NONE',  ( 18.83441953807343339, -276.9207081732492952, -322.8735580881307214 ) ) ;
#18344=CARTESIAN_POINT ( 'NONE',  ( -14.06544176718584538, -274.3626910399229928, -201.1714092339545914 ) ) ;
#18345=CARTESIAN_POINT ( 'NONE',  ( 26.68011411646424236, -273.9150457479317993, -228.1390880640642251 ) ) ;
#18347=CARTESIAN_POINT ( 'NONE',  ( -41.74507514058172575, -271.9966447099766924, -195.4400708904660178 ) ) ;
#18348=CARTESIAN_POINT ( 'NONE',  ( 19.10674449089164284, -295.6836344961678265, -321.9375228146101904 ) ) ;
#18351=CARTESIAN_POINT ( 'NONE',  ( 10.11924011719783678, -283.4596903078389118, -326.2999295594663636 ) ) ;
#18352=CARTESIAN_POINT ( 'NONE',  ( 24.29858650906719575, -283.9095344624773816, -314.8179868824415166 ) ) ;
#18353=CARTESIAN_POINT ( 'NONE',  ( -108.1940675032278989, -283.6635518405900598, -288.3565258922605494 ) ) ;
#18354=CARTESIAN_POINT ( 'NONE',  ( -4.730722392483621697, -275.0152028402754354, -336.5791208309219087 ) ) ;
#18355=CARTESIAN_POINT ( 'NONE',  ( -51.22607520076802956, -285.0917998893116305, -343.3387975395382341 ) ) ;
#18356=CARTESIAN_POINT ( 'NONE',  ( -70.78458020693736330, -275.9815293573620352, -336.0290822138302360 ) ) ;
#18357=CARTESIAN_POINT ( 'NONE',  ( 7.509228036664423733, -275.7603803280447323, -212.3730130350662648 ) ) ;
#18359=CARTESIAN_POINT ( 'NONE',  ( -79.83002468411946495, -280.2965779664895649, -206.2746259123988182 ) ) ;
#18362=CARTESIAN_POINT ( 'NONE',  ( -113.1056973315731966, -286.4170123369935936, -270.0115389209612999 ) ) ;
#18363=CARTESIAN_POINT ( 'NONE',  ( -58.46460753996408499, -294.5295006818424781, -340.4069923010587786 ) ) ;
#18364=CARTESIAN_POINT ( 'NONE',  ( -85.10785998166716126, -289.0402029797772343, -330.6927059614688460 ) ) ;
#18365=CARTESIAN_POINT ( 'NONE',  ( 32.80808305380109857, -285.4827918182606368, -246.7606533143973309 ) ) ;
#18366=CARTESIAN_POINT ( 'NONE',  ( -41.33691636436198991, -284.5756255925609253, -196.8678193536470644 ) ) ;
#18367=CARTESIAN_POINT ( 'NONE',  ( -93.30825996101474118, -289.4727319290576020, -221.9285029829443943 ) ) ;
#18368=CARTESIAN_POINT ( 'NONE',  ( -109.8884489380969995, -285.6067999126984773, -281.8267593677636000 ) ) ;
#18369=CARTESIAN_POINT ( 'NONE',  ( 35.29523946558853709, -273.7919793457811011, -289.0393314526837116 ) ) ;
#18370=CARTESIAN_POINT ( 'NONE',  ( 37.77176312748893139, -285.7890140262398972, -257.4620678854868743 ) ) ;
#18371=CARTESIAN_POINT ( 'NONE',  ( -4.530601066288855172, -300.4630443658264198, -195.3499233714474883 ) ) ;
#18372=CARTESIAN_POINT ( 'NONE',  ( 37.26752328373940770, -285.6744022905064639, -279.9160227446806175 ) ) ;
#18374=CARTESIAN_POINT ( 'NONE',  ( 35.75397222753428395, -282.4339738131332069, -265.8410371840897142 ) ) ;
#18375=CARTESIAN_POINT ( 'NONE',  ( -96.69588962739648252, -291.9213121728802776, -316.4817057893731089 ) ) ;
#18378=CARTESIAN_POINT ( 'NONE',  ( -81.01900643457557294, -297.5599272582323351, -332.0821831314446513 ) ) ;
#18380=CARTESIAN_POINT ( 'NONE',  ( -93.69480426405918649, -277.2397834031085040, -220.8509003234753152 ) ) ;
#18381=CARTESIAN_POINT ( 'NONE',  ( -61.62783006586693091, -290.9417541253687318, -197.4055430577087122 ) ) ;
#18382=CARTESIAN_POINT ( 'NONE',  ( -109.6728350530508749, -294.7600250780283204, -285.0749835905743339 ) ) ;
#18383=CARTESIAN_POINT ( 'NONE',  ( 22.20171578081307828, -280.8358549310615899, -313.4619473941257866 ) ) ;
#18384=CARTESIAN_POINT ( 'NONE',  ( 6.035317756951685375, -272.7251112422953838, -209.8015384451072975 ) ) ;
#18385=CARTESIAN_POINT ( 'NONE',  ( 23.34964704074147335, -295.4412049857933766, -311.8965365310359061 ) ) ;
#18386=CARTESIAN_POINT ( 'NONE',  ( -114.2704648735229114, -299.0519495502701943, -270.3937649182068981 ) ) ;
#18387=CARTESIAN_POINT ( 'NONE',  ( -113.2750847673237473, -271.2343597877220418, -261.8330824893644149 ) ) ;
#18388=CARTESIAN_POINT ( 'NONE',  ( -37.70690519882273861, -293.2964959873205544, -346.3598162958504645 ) ) ;
#18389=CARTESIAN_POINT ( 'NONE',  ( 0.1941150956643828696, -293.9878825109966556, -207.0646923910180703 ) ) ;
#18391=CARTESIAN_POINT ( 'NONE',  ( 28.88033943207292964, -293.9343733726302617, -239.1410542765987941 ) ) ;
#18393=CARTESIAN_POINT ( 'NONE',  ( -31.78331882588462776, -281.0024623258355518, -345.5240273004843630 ) ) ;
#18394=CARTESIAN_POINT ( 'NONE',  ( -72.12457855193380851, -295.5257536212666878, -334.5560021791729923 ) ) ;
#18395=CARTESIAN_POINT ( 'NONE',  ( -38.73254726487297717, -283.0691454756642429, -347.3485555567647793 ) ) ;
#18396=CARTESIAN_POINT ( 'NONE',  ( -113.1169260718744880, -284.0455835643530804, -284.2133555584199485 ) ) ;
#18397=CARTESIAN_POINT ( 'NONE',  ( -87.98845329025873241, -287.7618270266485752, -325.5216806314459177 ) ) ;
#18398=CARTESIAN_POINT ( 'NONE',  ( -31.70697657339797360, -281.4621583456681719, -346.4726083548007978 ) ) ;
#18399=CARTESIAN_POINT ( 'NONE',  ( 37.52018884129815035, -286.6822969570134205, -287.0700498393146631 ) ) ;
#18401=CARTESIAN_POINT ( 'NONE',  ( -28.78319214298199924, -296.5421137496775259, -343.7147542609420725 ) ) ;
#18402=CARTESIAN_POINT ( 'NONE',  ( -42.74624004448296688, -278.5443619850103119, -346.5805199832682320 ) ) ;
#18403=CARTESIAN_POINT ( 'NONE',  ( -107.9919616646128020, -278.4630570509071390, -251.8559034820763145 ) ) ;
#18404=CARTESIAN_POINT ( 'NONE',  ( 36.28635803359426149, -293.4358472490957297, -247.8242802307763668 ) ) ;
#18405=CARTESIAN_POINT ( 'NONE',  ( -78.39818155954780821, -281.6799034817786378, -333.7935980615562244 ) ) ;
#18407=CARTESIAN_POINT ( 'NONE',  ( 18.66424552418422067, -291.9426537540517756, -223.1727454704056299 ) ) ;
#18408=CARTESIAN_POINT ( 'NONE',  ( -112.3378101070132118, -294.5618006904203980, -269.5968316089573023 ) ) ;
#18409=ORIENTED_EDGE ( 'NONE', *, *, #36263, .F. ) ;
#18410=CARTESIAN_POINT ( 'NONE',  ( 18.87643636612662590, -293.7211003753546947, -317.0249109163572143 ) ) ;
#18412=CARTESIAN_POINT ( 'NONE',  ( -67.74223827176246004, -292.9809262143061233, -333.4151289067050357 ) ) ;
#18413=CARTESIAN_POINT ( 'NONE',  ( -105.4610463756093282, -272.2102085557035593, -234.6945883984020895 ) ) ;
#18414=CARTESIAN_POINT ( 'NONE',  ( 37.95797195979628924, -279.5793392145899929, -261.5180435393053244 ) ) ;
#18415=CARTESIAN_POINT ( 'NONE',  ( 25.13266511648668455, -288.2788703601202656, -226.1768802954254056 ) ) ;
#18416=CARTESIAN_POINT ( 'NONE',  ( -10.72607798969518100, -288.5285787855301010, -338.3903922582085784 ) ) ;
#18417=CARTESIAN_POINT ( 'NONE',  ( -109.9660872728296823, -279.9078790343306764, -282.9418373914640483 ) ) ;
#18418=CARTESIAN_POINT ( 'NONE',  ( -35.13193294281806089, -299.8403252642999064, -196.3471044052115531 ) ) ;
#18419=CARTESIAN_POINT ( 'NONE',  ( -41.89647546744252082, -275.9057098341030496, -343.6293937646144059 ) ) ;
#18421=CARTESIAN_POINT ( 'NONE',  ( -46.12324694399156755, -297.6103718778445568, -193.8847900960857373 ) ) ;
#18422=CARTESIAN_POINT ( 'NONE',  ( -106.4407881742127415, -292.1072631825048802, -298.1874343066943993 ) ) ;
#18423=CARTESIAN_POINT ( 'NONE',  ( 38.91105295877255088, -295.1513832562801554, -270.2901514668143363 ) ) ;
#18426=CARTESIAN_POINT ( 'NONE',  ( -95.20014861465652700, -291.8317314030039711, -225.6812275701722967 ) ) ;
#18429=CARTESIAN_POINT ( 'NONE',  ( 37.11581992329399782, -291.5136227898073571, -256.3474392927533927 ) ) ;
#18430=CARTESIAN_POINT ( 'NONE',  ( -34.76457602019346638, -298.4168711406839520, -193.3821205562305749 ) ) ;
#18434=CARTESIAN_POINT ( 'NONE',  ( -88.20189736861073015, -292.8751920107506521, -213.4757236552805466 ) ) ;
#18435=CARTESIAN_POINT ( 'NONE',  ( 13.79469577742117714, -289.1948066931273615, -206.1857440867352693 ) ) ;
#18436=CARTESIAN_POINT ( 'NONE',  ( -90.99463444515654942, -287.2888084190585118, -218.1197759237803382 ) ) ;
#18437=CARTESIAN_POINT ( 'NONE',  ( 29.51023075727174572, -273.1067905951841226, -236.7330380446502716 ) ) ;
#18438=CARTESIAN_POINT ( 'NONE',  ( -11.00315423067759291, -276.3181981698037362, -200.6813397741311462 ) ) ;
#18440=CARTESIAN_POINT ( 'NONE',  ( -82.58524743923179301, -289.5088510396396373, -211.1830014874893493 ) ) ;
#18441=CARTESIAN_POINT ( 'NONE',  ( -71.00047182164078663, -279.3519837230407461, -338.2388947022027423 ) ) ;
#18443=CARTESIAN_POINT ( 'NONE',  ( -70.94166808009228475, -279.5959073069824967, -205.5392982787042513 ) ) ;
#18444=CARTESIAN_POINT ( 'NONE',  ( 29.40414618432475180, -281.3031394763017943, -300.2995432541271157 ) ) ;
#18445=CARTESIAN_POINT ( 'NONE',  ( -38.52634079958206570, -278.1463461582590071, -347.0428572528606992 ) ) ;
#18446=CARTESIAN_POINT ( 'NONE',  ( 36.80359155852602981, -280.5892394684449869, -289.6090903544763364 ) ) ;
#18447=CARTESIAN_POINT ( 'NONE',  ( 199.7552170467075712, 291.4512671170426188, -82.50257151101990871 ) ) ;
#18448=CARTESIAN_POINT ( 'NONE',  ( 7.089010765944712134, -275.5818951274637243, -207.6961129891504640 ) ) ;
#18449=CARTESIAN_POINT ( 'NONE',  ( -92.68278473143705298, -274.7969085751452667, -217.8056560969009183 ) ) ;
#18450=CARTESIAN_POINT ( 'NONE',  ( -109.1418805571601069, -281.0519495502701943, -270.3937649182068412 ) ) ;
#18452=CARTESIAN_POINT ( 'NONE',  ( 132.9888089158688445, -299.5541904835127980, -195.3611179825600175 ) ) ;
#18453=CARTESIAN_POINT ( 'NONE',  ( -74.86234805680348359, -290.6440936569449605, -333.3554419440064294 ) ) ;
#18454=CARTESIAN_POINT ( 'NONE',  ( 9.172542058821463229, -288.4412471137406442, -210.2745197673373525 ) ) ;
#18455=CARTESIAN_POINT ( 'NONE',  ( -61.29623385734826968, -288.7202146284037667, -339.4268329349933992 ) ) ;
#18456=CARTESIAN_POINT ( 'NONE',  ( -52.15528865565833172, -285.3751840040727075, -194.8078682744807963 ) ) ;
#18458=CARTESIAN_POINT ( 'NONE',  ( -38.92242558352145920, -281.4721431534111957, -344.1568175633397004 ) ) ;
#18459=CARTESIAN_POINT ( 'NONE',  ( -26.26761788924477159, -290.7702737032774394, -343.8175978330015141 ) ) ;
#18460=CARTESIAN_POINT ( 'NONE',  ( -98.11500255970440776, -282.4562482126055443, -312.1311791736333703 ) ) ;
#18461=CARTESIAN_POINT ( 'NONE',  ( -99.89622763267232131, -280.3968329430364861, -231.6871321728701787 ) ) ;
#18463=CARTESIAN_POINT ( 'NONE',  ( -37.80386070040891866, -277.5504071699263022, -343.4336584521614100 ) ) ;
#18464=CARTESIAN_POINT ( 'NONE',  ( -112.2484377030699392, -289.5493506667588122, -254.2684024630390525 ) ) ;
#18465=CARTESIAN_POINT ( 'NONE',  ( -64.49970297386390428, -286.5093623257991453, -198.4679023020324564 ) ) ;
#18466=CARTESIAN_POINT ( 'NONE',  ( -68.48160212870322994, -286.1462142809880902, -199.9917000953179524 ) ) ;
#18467=CARTESIAN_POINT ( 'NONE',  ( -78.37487713596070193, -283.7883067704338487, -330.7372588755456491 ) ) ;
#18470=CARTESIAN_POINT ( 'NONE',  ( -95.42856207035013938, -291.7469979246462799, -319.0250604810841537 ) ) ;
#18471=CARTESIAN_POINT ( 'NONE',  ( 25.30118074852753907, -292.8218021461206604, -314.3062669074489008 ) ) ;
#18472=CARTESIAN_POINT ( 'NONE',  ( 7.484358705474618567, -273.7397821557955240, -212.4471050251708846 ) ) ;
#18473=CARTESIAN_POINT ( 'NONE',  ( -95.50983521154761036, -295.2203989268954842, -320.6580448047077994 ) ) ;
#18474=CARTESIAN_POINT ( 'NONE',  ( -47.06698309518480272, -290.4062500512792440, -197.3123218074406964 ) ) ;
#18475=CARTESIAN_POINT ( 'NONE',  ( -97.24153419482951222, -294.1917087564575581, -313.8567035752797665 ) ) ;
#18476=CARTESIAN_POINT ( 'NONE',  ( -101.9856345685396661, -291.2844843612261343, -305.2293317523063365 ) ) ;
#18478=CARTESIAN_POINT ( 'NONE',  ( 31.65196417039437549, -291.1625969193617038, -240.5298808247407294 ) ) ;
#18479=CARTESIAN_POINT ( 'NONE',  ( 29.77500962608763402, -295.1091140089343412, -236.7746029264955610 ) ) ;
#18480=CARTESIAN_POINT ( 'NONE',  ( 27.86218812237793685, -288.0404830029386289, -236.9047559861107004 ) ) ;
#18481=CARTESIAN_POINT ( 'NONE',  ( 18.79336908817745311, -276.8345957236899153, -220.0125979619869270 ) ) ;
#18482=CARTESIAN_POINT ( 'NONE',  ( -42.79330527075682511, -275.9144385164120195, -346.7698132997780931 ) ) ;
#18483=CARTESIAN_POINT ( 'NONE',  ( -106.3637795446746139, -296.1838346164104223, -236.5955826987196815 ) ) ;
#18484=CARTESIAN_POINT ( 'NONE',  ( 35.70358694253413034, -273.9512698972658882, -282.6016998127785769 ) ) ;
#18485=CARTESIAN_POINT ( 'NONE',  ( -77.58008269017265945, -277.5877919087350847, -207.6723184437707062 ) ) ;
#18486=CARTESIAN_POINT ( 'NONE',  ( -59.61064535139623644, -274.9624389552184880, -200.3706139979180421 ) ) ;
#18487=CARTESIAN_POINT ( 'NONE',  ( -67.41186304433895771, -275.8399085361755851, -340.3770141698942666 ) ) ;
#18489=CARTESIAN_POINT ( 'NONE',  ( -59.51444554745580717, -274.4088655965707630, -200.6499403494055116 ) ) ;
#18492=CARTESIAN_POINT ( 'NONE',  ( -29.18091182051923482, -286.9694728694363448, -345.3255032745319681 ) ) ;
#18493=CARTESIAN_POINT ( 'NONE',  ( -6.527050292322345015, -274.3018033424677355, -204.1836493090405895 ) ) ;
#18495=CARTESIAN_POINT ( 'NONE',  ( 32.86487654107115475, -287.9560881104892474, -301.9844731555711519 ) ) ;
#18496=CARTESIAN_POINT ( 'NONE',  ( -110.7629650729319195, -289.9261408980842702, -293.6667020781873134 ) ) ;
#18497=CARTESIAN_POINT ( 'NONE',  ( -112.5093130267115811, -274.5878523694335058, -267.5873348197950463 ) ) ;
#18498=CARTESIAN_POINT ( 'NONE',  ( -107.5163721759210489, -294.8918204388995150, -244.2205633017366040 ) ) ;
#18500=CARTESIAN_POINT ( 'NONE',  ( -2.454303412367441872, -279.6989473726712845, -201.8845450564031978 ) ) ;
#18503=CARTESIAN_POINT ( 'NONE',  ( -109.1708615965814033, -276.2734586993274775, -291.9824285362325895 ) ) ;
#18504=FACE_OUTER_BOUND ( 'NONE', #73551, .T. ) ;
#18505=CARTESIAN_POINT ( 'NONE',  ( -110.7646170361288114, -289.3723260364604357, -268.4361161895217265 ) ) ;
#18507=CARTESIAN_POINT ( 'NONE',  ( -110.6605081141568832, -288.7547481662529094, -254.5702013393155596 ) ) ;
#18508=CARTESIAN_POINT ( 'NONE',  ( -51.71546725106541942, -275.3851976807318351, -198.0308801878181839 ) ) ;
#18509=CARTESIAN_POINT ( 'NONE',  ( 37.67274262819614705, -282.7941619088899188, -255.8201526687256546 ) ) ;
#18510=CARTESIAN_POINT ( 'NONE',  ( 51.20065605406508524, -297.1753657202241925, -195.0356064417869959 ) ) ;
#18511=CARTESIAN_POINT ( 'NONE',  ( -84.86177938539310617, -283.7293326280835117, -325.7762970166370451 ) ) ;
#18512=CARTESIAN_POINT ( 'NONE',  ( -87.75003621855245228, -274.7568427906131205, -216.6781383874958351 ) ) ;
#18513=CARTESIAN_POINT ( 'NONE',  ( 30.32026780601015759, -275.9812329556879718, -242.3990187832259267 ) ) ;
#18514=CARTESIAN_POINT ( 'NONE',  ( -72.52545093352124184, -287.5939705805653261, -337.2442618739322597 ) ) ;
#18515=CARTESIAN_POINT ( 'NONE',  ( -73.29425776864243858, -285.5286868697865543, -336.2401334786221696 ) ) ;
#18517=CARTESIAN_POINT ( 'NONE',  ( -98.09166856217510144, -272.0415002934558970, -229.2380635246693714 ) ) ;
#18520=CARTESIAN_POINT ( 'NONE',  ( 15.47714442649860977, -294.1630452527837747, -326.3894114101727837 ) ) ;
#18521=CARTESIAN_POINT ( 'NONE',  ( -80.27548315869583462, -287.4478143251849360, -209.2358994350518913 ) ) ;
#18523=CARTESIAN_POINT ( 'NONE',  ( -99.86837403722181250, -270.6952119285918457, -220.4570493818173702 ) ) ;
#18524=CARTESIAN_POINT ( 'NONE',  ( -114.2160391143859357, -277.7697950614236220, -268.7274546917865337 ) ) ;
#18525=CARTESIAN_POINT ( 'NONE',  ( -103.1182682241300483, -288.4449194479786343, -308.9347854765167085 ) ) ;
#18526=CARTESIAN_POINT ( 'NONE',  ( -38.88032747611086393, -284.5918887233277133, -344.0509995412723470 ) ) ;
#18527=CARTESIAN_POINT ( 'NONE',  ( -74.50293818045901162, -279.3139269816320507, -334.3690581167077767 ) ) ;
#18528=CARTESIAN_POINT ( 'NONE',  ( -102.0293772130001742, -286.5140770273969224, -229.6903579021214910 ) ) ;
#18529=CARTESIAN_POINT ( 'NONE',  ( 3.779841757612731890, -282.6053565897504996, -207.5770524743816452 ) ) ;
#18530=CARTESIAN_POINT ( 'NONE',  ( -21.35686202443334736, -274.4184003559284406, -195.0385784921492984 ) ) ;
#18531=CARTESIAN_POINT ( 'NONE',  ( -20.12816954715411910, -276.6703201100349361, -345.4671147148210366 ) ) ;
#18532=CARTESIAN_POINT ( 'NONE',  ( -35.59274164050663103, -296.9502258989028292, -344.7933157173953873 ) ) ;
#18536=CARTESIAN_POINT ( 'NONE',  ( -86.64028556492256428, -295.5154585552031676, -212.7597672193894027 ) ) ;
#18537=CARTESIAN_POINT ( 'NONE',  ( -40.51470909172113721, -276.6007421237648032, -343.3661982498928182 ) ) ;
#18538=CARTESIAN_POINT ( 'NONE',  ( -112.6806232171716147, -273.9350040771517456, -256.2192089527511598 ) ) ;
#18539=CARTESIAN_POINT ( 'NONE',  ( -46.87733123603825192, -287.6897051722824585, -196.9131398999693090 ) ) ;
#18540=CARTESIAN_POINT ( 'NONE',  ( -58.63907948225442368, -296.8426682684632851, -343.6905287430371914 ) ) ;
#18541=CARTESIAN_POINT ( 'NONE',  ( -113.7261772695988498, -297.8382084821406011, -263.9192050118442694 ) ) ;
#18542=CARTESIAN_POINT ( 'NONE',  ( -111.9482925418126200, -292.4692947655991588, -276.8126949973831188 ) ) ;
#18543=CARTESIAN_POINT ( 'NONE',  ( -95.34582016535756566, -277.2049161315813421, -223.0795096187027582 ) ) ;
#18544=CARTESIAN_POINT ( 'NONE',  ( -107.8157848462118267, -280.7865802559705344, -246.2293998910118944 ) ) ;
#18545=CARTESIAN_POINT ( 'NONE',  ( -109.5242528875122758, -270.8201157981344522, -251.1493279800756682 ) ) ;
#18546=CARTESIAN_POINT ( 'NONE',  ( -108.1401228059177413, -286.0638054887901376, -297.4866024634024484 ) ) ;
#18547=CARTESIAN_POINT ( 'NONE',  ( 30.76729199987585517, -286.8354246339021074, -297.6160624550819875 ) ) ;
#18548=CARTESIAN_POINT ( 'NONE',  ( 86.20037202169200441, 82.24261404803831965, -301.9681809940666426 ) ) ;
#18550=CARTESIAN_POINT ( 'NONE',  ( -7.003848871517688757, -286.1282589226604500, -203.9267403824592009 ) ) ;
#18552=CARTESIAN_POINT ( 'NONE',  ( -18.97902861234918603, -283.9009467438962133, -344.8759460500657497 ) ) ;
#18553=CARTESIAN_POINT ( 'NONE',  ( -36.74015813344699666, -274.3931973679943894, -197.3300331140614503 ) ) ;
#18554=CARTESIAN_POINT ( 'NONE',  ( -4.927943124689051047, -285.2644750169177428, -200.9539348009649302 ) ) ;
#18556=CARTESIAN_POINT ( 'NONE',  ( -14.30981169128479635, -281.2848034912624939, -197.0773072859016395 ) ) ;
#18558=CARTESIAN_POINT ( 'NONE',  ( -17.19385563167945463, -281.8277685797074241, -196.7623943987474888 ) ) ;
#18559=CARTESIAN_POINT ( 'NONE',  ( 6.168808037376875220, -280.9585432400838840, -206.8585198417224262 ) ) ;
#18560=CARTESIAN_POINT ( 'NONE',  ( -102.0172624299487154, -288.4809262143061801, -239.1787733560258289 ) ) ;
#18561=CARTESIAN_POINT ( 'NONE',  ( -103.5911469518875379, -256.6625002471756147, -326.7956433880881377 ) ) ;
#18564=CARTESIAN_POINT ( 'NONE',  ( 20.39755320262476346, -276.8941315215337227, -222.7564222560362452 ) ) ;
#18565=CARTESIAN_POINT ( 'NONE',  ( 24.83231157103504927, -22.65643835391063021, -344.9118043155972373 ) ) ;
#18567=CARTESIAN_POINT ( 'NONE',  ( 30.80602539222534020, -279.9748742791759923, -300.9466636241256765 ) ) ;
#18568=CARTESIAN_POINT ( 'NONE',  ( 28.58519336549668566, -294.8148115627031416, -232.5772758524784365 ) ) ;
#18569=CARTESIAN_POINT ( 'NONE',  ( -78.01333230909250460, -294.9630719902157807, -331.1652550965862929 ) ) ;
#18570=CARTESIAN_POINT ( 'NONE',  ( -84.22388375057433052, -290.9347692804208236, -209.2891578344852519 ) ) ;
#18571=CARTESIAN_POINT ( 'NONE',  ( 82.64890176555634582, -297.1582149144751384, -195.3611179825600175 ) ) ;
#18573=CARTESIAN_POINT ( 'NONE',  ( -109.7928274324748799, -294.8188106286953030, -294.6395125900769472 ) ) ;
#18574=CARTESIAN_POINT ( 'NONE',  ( 36.42873542136356235, -285.9971159549807567, -273.8173957554118942 ) ) ;
#18575=CARTESIAN_POINT ( 'NONE',  ( 13.73616695035188506, -294.6377686880034048, -216.4916742013536748 ) ) ;
#18576=CARTESIAN_POINT ( 'NONE',  ( -107.8604164539242305, -285.5948094133122481, -291.1027325633305622 ) ) ;
#18578=CARTESIAN_POINT ( 'NONE',  ( 21.12343286581323554, -293.8204302666478611, -220.5952018966825960 ) ) ;
#18580=CARTESIAN_POINT ( 'NONE',  ( -48.33175769892876161, -283.6881636979160817, -342.5913545605537252 ) ) ;
#18581=CARTESIAN_POINT ( 'NONE',  ( -110.4296214064108455, -295.6387926320588804, -247.2471196708307559 ) ) ;
#18582=CARTESIAN_POINT ( 'NONE',  ( -114.0273298749362567, -291.4157025437480684, -265.5162226897136293 ) ) ;
#18583=CARTESIAN_POINT ( 'NONE',  ( -44.89724817652989941, -292.4514122476036846, -193.7416616088525529 ) ) ;
#18584=CARTESIAN_POINT ( 'NONE',  ( -86.72781777403862691, -289.9283186857657029, -324.1885169088473617 ) ) ;
#18587=CARTESIAN_POINT ( 'NONE',  ( -97.28247472248484939, -297.7838843707907586, -316.7012628366149443 ) ) ;
#18588=CARTESIAN_POINT ( 'NONE',  ( -113.9446275073758841, -271.3472703805991273, -270.3458084817817735 ) ) ;
#18589=CARTESIAN_POINT ( 'NONE',  ( -62.37815739355075095, -278.7771840396258654, -201.4847457254723793 ) ) ;
#18592=CARTESIAN_POINT ( 'NONE',  ( 9.477860672189608593, -274.1843785355497403, -209.3082259173498869 ) ) ;
#18593=CARTESIAN_POINT ( 'NONE',  ( -82.35243724732998771, -295.9052413621246274, -211.9462956158240559 ) ) ;
#18594=CARTESIAN_POINT ( 'NONE',  ( 20.15304636032786689, -278.0665701533766878, -317.3409233854697504 ) ) ;
#18595=CARTESIAN_POINT ( 'NONE',  ( 26.34754225808038441, -273.1747192196713172, -232.1229909113000360 ) ) ;
#18596=CARTESIAN_POINT ( 'NONE',  ( -55.88890868371046139, -296.5012793220153071, -341.4287923844375996 ) ) ;
#18597=CARTESIAN_POINT ( 'NONE',  ( -96.35730656854710219, -298.2390007016339268, -226.8498718945271264 ) ) ;
#18599=CARTESIAN_POINT ( 'NONE',  ( -67.87580672487833056, -299.2582721280604119, -200.4900846345941261 ) ) ;
#18601=CARTESIAN_POINT ( 'NONE',  ( 6.674283129644242862, -296.6017529348180801, -195.2094072685388255 ) ) ;
#18602=CARTESIAN_POINT ( 'NONE',  ( 30.68345933375126222, -294.5626650876890267, -297.2666195342657716 ) ) ;
#18603=CARTESIAN_POINT ( 'NONE',  ( -92.09956273180337405, -289.8250576462705226, -221.1797759443949758 ) ) ;
#18604=CARTESIAN_POINT ( 'NONE',  ( 17.53318101573682242, -300.7392505651913552, -195.3424018486777527 ) ) ;
#18605=CARTESIAN_POINT ( 'NONE',  ( 32.96607768530838456, -276.4436151914591733, -301.6076102977514779 ) ) ;
#18606=CARTESIAN_POINT ( 'NONE',  ( -96.28262770702696116, -273.3229362806323479, -227.2078027785737788 ) ) ;
#18607=CARTESIAN_POINT ( 'NONE',  ( 24.59315650731292635, -284.1116823501766362, -313.3079452837239955 ) ) ;
#18608=CARTESIAN_POINT ( 'NONE',  ( -13.59102928407611799, -281.4349390235323085, -343.0880312014667197 ) ) ;
#18610=CARTESIAN_POINT ( 'NONE',  ( -95.13966416192549502, -277.2134565693370973, -321.0829884165950148 ) ) ;
#18612=CARTESIAN_POINT ( 'NONE',  ( -107.5497577288777507, -283.4771448171619568, -290.9832934294973370 ) ) ;
#18613=CARTESIAN_POINT ( 'NONE',  ( 18.40626901811734584, -280.2540963079276253, -320.8573954732515290 ) ) ;
#18614=EDGE_CURVE ( 'NONE', #71727, #43403, #19914, .T. ) ;
#18615=CARTESIAN_POINT ( 'NONE',  ( 33.45984166988934305, -274.3905349517042964, -290.4700070139122658 ) ) ;
#18616=CARTESIAN_POINT ( 'NONE',  ( -62.21566128194445611, -279.3756608151099954, -341.1700691521882618 ) ) ;
#18619=CARTESIAN_POINT ( 'NONE',  ( -35.83038556322976831, -296.3106919061331155, -194.3748902813860866 ) ) ;
#18620=CARTESIAN_POINT ( 'NONE',  ( -68.23796041456832029, -279.4571092230173122, -338.8985272977748195 ) ) ;
#18622=CARTESIAN_POINT ( 'NONE',  ( -107.9484528984091867, -286.1235339959541193, -297.4140488612280251 ) ) ;
#18623=ORIENTED_EDGE ( 'NONE', *, *, #12440, .F. ) ;
#18625=CARTESIAN_POINT ( 'NONE',  ( 17.99197929496902049, -284.8448689015404511, -219.7144744771975127 ) ) ;
#18627=CARTESIAN_POINT ( 'NONE',  ( -105.3354824887800305, -294.9788323073088350, -298.0012349176078601 ) ) ;
#18628=CARTESIAN_POINT ( 'NONE',  ( 1.945534855811330122, -286.6598616586912271, -333.3482487854449232 ) ) ;
#18630=CARTESIAN_POINT ( 'NONE',  ( -108.5992076279081004, -294.8561388165281869, -246.8007446595710235 ) ) ;
#18631=CARTESIAN_POINT ( 'NONE',  ( 9.401446153870715250, -285.1615118574719645, -210.0470563836351801 ) ) ;
#18632=CARTESIAN_POINT ( 'NONE',  ( 36.14698507957970008, -283.0569138900773396, -263.0520707572362085 ) ) ;
#18633=CARTESIAN_POINT ( 'NONE',  ( -52.73454351943054519, -281.4864868028225828, -344.8261480084637469 ) ) ;
#18634=CARTESIAN_POINT ( 'NONE',  ( -82.54626709963542908, -289.6897868643849847, -327.6808102786136487 ) ) ;
#18636=CARTESIAN_POINT ( 'NONE',  ( -102.6873955946119565, -280.4352975536023678, -236.4076610719573068 ) ) ;
#18637=CARTESIAN_POINT ( 'NONE',  ( 30.16656945971872972, -281.9775348375103476, -242.1612019583262736 ) ) ;
#18638=CARTESIAN_POINT ( 'NONE',  ( 32.52697351381365820, -289.8998175570631588, -298.7274278242689434 ) ) ;
#18641=CARTESIAN_POINT ( 'NONE',  ( -104.2295303334646945, -273.0487839751910997, -232.1094138764649415 ) ) ;
#18642=CARTESIAN_POINT ( 'NONE',  ( -96.43155670463150386, -293.1599954154496572, -224.7515174997466829 ) ) ;
#18643=DIRECTION ( 'NONE',  ( -1.000000000000000000, -0.000000000000000000, -0.000000000000000000 ) ) ;
#18644=CARTESIAN_POINT ( 'NONE',  ( 25.18497378105907814, -295.4090924074130839, -220.4570493818173702 ) ) ;
#18646=CARTESIAN_POINT ( 'NONE',  ( 28.91473217082226554, -274.0232732294889502, -305.9690302599933034 ) ) ;
#18648=CARTESIAN_POINT ( 'NONE',  ( -39.10991420598376322, -293.4738731897464277, -346.5406023381209479 ) ) ;
#18649=CARTESIAN_POINT ( 'NONE',  ( -40.51437295184805265, -297.5188686772299320, -197.3559385014798977 ) ) ;
#18651=CARTESIAN_POINT ( 'NONE',  ( 32.05879219835336613, -289.3991662531844895, -295.1457788952432111 ) ) ;
#18652=CARTESIAN_POINT ( 'NONE',  ( 31.28234780054427944, -283.6784855533242649, -298.0868110734988363 ) ) ;
#18653=CARTESIAN_POINT ( 'NONE',  ( -109.8773459360917997, -292.2840325697873709, -246.1707123410854763 ) ) ;
#18654=CARTESIAN_POINT ( 'NONE',  ( -47.69335392109125138, -293.2384739100841671, -194.5043583501977764 ) ) ;
#18655=CARTESIAN_POINT ( 'NONE',  ( -64.06963382229783122, -291.5268855571030144, -202.4166086296711740 ) ) ;
#18656=CARTESIAN_POINT ( 'NONE',  ( -99.01468426797714528, -287.1312837319169375, -227.6600314654222927 ) ) ;
#18657=CARTESIAN_POINT ( 'NONE',  ( -68.67446841571224070, -279.8182932477030818, -200.0099874910655444 ) ) ;
#18658=CARTESIAN_POINT ( 'NONE',  ( -109.8407719097109521, -294.3593574740602890, -291.6952726328509016 ) ) ;
#18659=CARTESIAN_POINT ( 'NONE',  ( -71.74064495157217891, -283.3275090847915294, -339.2502506492066914 ) ) ;
#18660=CIRCLE ( 'NONE', #71609, 1.000000000000000888 ) ;
#18661=CARTESIAN_POINT ( 'NONE',  ( 35.83938354246152613, -277.2498857938909964, -257.8200225499571161 ) ) ;
#18662=CARTESIAN_POINT ( 'NONE',  ( -21.39648532958013050, -282.7662352645559167, -200.3538533559491555 ) ) ;
#18663=CARTESIAN_POINT ( 'NONE',  ( -38.54941638853789954, -275.2067345497992505, -346.1162953996163765 ) ) ;
#18665=CARTESIAN_POINT ( 'NONE',  ( 5.623224251494886694, -281.9598166007838245, -329.4542962228417196 ) ) ;
#18667=CARTESIAN_POINT ( 'NONE',  ( -101.5667326911130175, -280.3094560961239949, -228.5140120107250254 ) ) ;
#18668=CARTESIAN_POINT ( 'NONE',  ( 34.84709516768052140, -286.9433776802270586, -296.6231371575196931 ) ) ;
#18669=CARTESIAN_POINT ( 'NONE',  ( 34.62793203682779364, -295.0868981206335206, -253.0343474516622564 ) ) ;
#18670=CARTESIAN_POINT ( 'NONE',  ( 37.40168358230796741, -277.3396654041292209, -285.1890311517540795 ) ) ;
#18671=CARTESIAN_POINT ( 'NONE',  ( 37.70194245288274004, -277.0547571151574289, -285.2523900011760247 ) ) ;
#18672=CARTESIAN_POINT ( 'NONE',  ( -8.740633481064914889, -276.5005435795611106, -337.5384822809604657 ) ) ;
#18673=CARTESIAN_POINT ( 'NONE',  ( -96.20001071998778741, -297.9165606053701936, -316.5750520847586245 ) ) ;
#18674=CARTESIAN_POINT ( 'NONE',  ( -99.61902232865598705, -283.1138997044207031, -228.8693890952451397 ) ) ;
#18675=CARTESIAN_POINT ( 'NONE',  ( -19.38758490519804312, -291.9436003450615544, -195.4504883300527638 ) ) ;
#18676=CARTESIAN_POINT ( 'NONE',  ( -15.16539300411809776, -290.3699287529752837, -343.3179531839842298 ) ) ;
#18679=CARTESIAN_POINT ( 'NONE',  ( 6.873573640867734369, -291.5905150399097465, -211.8868874343441178 ) ) ;
#18681=CARTESIAN_POINT ( 'NONE',  ( -88.24335383574977243, -289.9302719649409710, -213.3731548560725173 ) ) ;
#18682=CARTESIAN_POINT ( 'NONE',  ( -60.26157742424427965, -291.4135099391671702, -200.9772142064452396 ) ) ;
#18684=CARTESIAN_POINT ( 'NONE',  ( -70.49295314886026631, -290.5585967235142562, -339.5310717999277585 ) ) ;
#18685=CARTESIAN_POINT ( 'NONE',  ( -103.3907855263951490, -279.3074695478624676, -239.1037614368844686 ) ) ;
#18687=CARTESIAN_POINT ( 'NONE',  ( -110.9227162735125916, -295.1997044258587266, -292.0252043671100637 ) ) ;
#18688=CARTESIAN_POINT ( 'NONE',  ( -36.57479149920327899, -286.7129501317197651, -193.4538532475847603 ) ) ;
#18689=CARTESIAN_POINT ( 'NONE',  ( 38.08841996104084870, -288.0776278303706022, -285.7247528051314589 ) ) ;
#18690=CARTESIAN_POINT ( 'NONE',  ( -110.4115472345471574, -284.8781483011757132, -270.9136937307862354 ) ) ;
#18691=CARTESIAN_POINT ( 'NONE',  ( -104.5909623734863345, -255.9058999860209269, -326.6256074632946707 ) ) ;
#18692=CARTESIAN_POINT ( 'NONE',  ( 4.381996518072155844, -57.88619191719195101, -353.6676151370956518 ) ) ;
#18693=CARTESIAN_POINT ( 'NONE',  ( -63.40552176226377412, -182.3960580802271920, -358.6459566522576097 ) ) ;
#18694=CARTESIAN_POINT ( 'NONE',  ( 30.32806307829934767, -274.3758262439469604, -242.4178872203009689 ) ) ;
#18695=CARTESIAN_POINT ( 'NONE',  ( -35.12199346387371435, -275.9439523763949182, -343.6366185044350914 ) ) ;
#18696=CARTESIAN_POINT ( 'NONE',  ( -114.0589307625553630, -296.1410589333410712, -263.8694035640912148 ) ) ;
#18697=CARTESIAN_POINT ( 'NONE',  ( 122.5836672862912309, 147.2107594463095381, -260.7345742909203636 ) ) ;
#18698=CARTESIAN_POINT ( 'NONE',  ( 16.59559936688325621, -274.9897309909188721, -324.6943247859525172 ) ) ;
#18699=CARTESIAN_POINT ( 'NONE',  ( -63.68810199495433721, -275.4641019763753320, -201.1821179894019451 ) ) ;
#18700=CARTESIAN_POINT ( 'NONE',  ( -26.26400523166820022, -299.1289105048854253, -193.5946887281719455 ) ) ;
#18701=CARTESIAN_POINT ( 'NONE',  ( -42.66214133136008968, -289.6132901962125175, -343.2793248315861661 ) ) ;
#18702=CARTESIAN_POINT ( 'NONE',  ( -86.28458531810886711, -296.5145445294927526, -329.5958443622394043 ) ) ;
#18703=CARTESIAN_POINT ( 'NONE',  ( -98.18916324516062843, -297.6738231037157334, -223.2536223037349146 ) ) ;
#18704=CARTESIAN_POINT ( 'NONE',  ( -73.30055592941759812, -295.7100381190964526, -333.8903293264039576 ) ) ;
#18707=CARTESIAN_POINT ( 'NONE',  ( -28.74021323455523813, -278.8641874720310625, -345.4825186157805774 ) ) ;
#18709=CARTESIAN_POINT ( 'NONE',  ( 1.348456666218617261, -280.0618252109069317, -203.7978372947814307 ) ) ;
#18711=CARTESIAN_POINT ( 'NONE',  ( 3.274527898685858140, -277.4326124039857291, -331.3015025282545025 ) ) ;
#18712=CARTESIAN_POINT ( 'NONE',  ( -45.51800456970485698, -278.9144098953296975, -345.9589743188711850 ) ) ;
#18713=CARTESIAN_POINT ( 'NONE',  ( -110.5826439677304194, -276.3450621847935054, -288.1401053648218635 ) ) ;
#18714=CARTESIAN_POINT ( 'NONE',  ( -109.9476206690420526, -273.1518800605063007, -262.2144165637978972 ) ) ;
#18715=CARTESIAN_POINT ( 'NONE',  ( -93.17974848793016918, -295.8039727188680104, -222.4096305120141039 ) ) ;
#18717=CARTESIAN_POINT ( 'NONE',  ( -104.2705400919363399, -278.3254169924786652, -299.6344783160370184 ) ) ;
#18719=CARTESIAN_POINT ( 'NONE',  ( -3.295332338453454746, -287.2968809615135797, -338.8894685324717670 ) ) ;
#18720=CARTESIAN_POINT ( 'NONE',  ( -93.60348516543066921, -275.2416943134270468, -220.7666405177664330 ) ) ;
#18723=CARTESIAN_POINT ( 'NONE',  ( -109.0991129620712030, -289.5607162052871217, -284.6897228256451058 ) ) ;
#18725=CARTESIAN_POINT ( 'NONE',  ( -96.19765763992201357, -283.2332725913774425, -319.8717871418928098 ) ) ;
#18726=CARTESIAN_POINT ( 'NONE',  ( 29.05028276768653228, -280.2306043492196750, -303.1894127679742610 ) ) ;
#18727=CARTESIAN_POINT ( 'NONE',  ( 17.51406107999513395, -279.4307402858245837, -221.3078777209174746 ) ) ;
#18728=CARTESIAN_POINT ( 'NONE',  ( -44.13185445101422744, -284.0454626924659465, -196.2314477962858064 ) ) ;
#18729=CARTESIAN_POINT ( 'NONE',  ( 32.54108383381068137, -289.1964505211116716, -242.9922279296531258 ) ) ;
#18730=CARTESIAN_POINT ( 'NONE',  ( -98.33207288189734641, -280.3223544212774527, -229.4381993958763815 ) ) ;
#18732=CARTESIAN_POINT ( 'NONE',  ( -11.85742624963008218, -294.3839197310990698, -199.7689481161864364 ) ) ;
#18734=CARTESIAN_POINT ( 'NONE',  ( -69.51268503985730263, -277.8744631738266548, -201.5065117220206048 ) ) ;
#18735=CARTESIAN_POINT ( 'NONE',  ( -68.07273214200738209, -278.1180596106455027, -336.7035830925050846 ) ) ;
#18736=CARTESIAN_POINT ( 'NONE',  ( -93.93716410975736153, -285.8669174671474025, -319.8280957088907144 ) ) ;
#18740=CARTESIAN_POINT ( 'NONE',  ( -99.48216543947647494, -291.8937510049568118, -313.3480551792785036 ) ) ;
#18741=CARTESIAN_POINT ( 'NONE',  ( -99.21249642911720912, -293.9774479272222152, -312.7747351184175955 ) ) ;
#18743=CARTESIAN_POINT ( 'NONE',  ( -1.036807435070341565, -285.7187413196473358, -202.6402675199855139 ) ) ;
#18744=CARTESIAN_POINT ( 'NONE',  ( -108.8789730053623828, -289.1893774704858515, -252.1753094629680163 ) ) ;
#18746=CARTESIAN_POINT ( 'NONE',  ( 36.08060790628862691, -274.1814927167730502, -266.1271425914335396 ) ) ;
#18747=CARTESIAN_POINT ( 'NONE',  ( 20.64398495721016502, -292.3358468826331773, -316.7335665964382088 ) ) ;
#18748=CARTESIAN_POINT ( 'NONE',  ( 202.9737475146022803, 296.4636489462809550, -68.70538243550777224 ) ) ;
#18750=CARTESIAN_POINT ( 'NONE',  ( -53.22592131223413503, -290.3320553694580326, -195.6720060197304747 ) ) ;
#18751=CARTESIAN_POINT ( 'NONE',  ( -93.88098580630865797, -286.8185093421110423, -222.9295926848291742 ) ) ;
#18752=CARTESIAN_POINT ( 'NONE',  ( 28.02053394467954206, -286.3036576663770347, -309.1135678290094688 ) ) ;
#18753=CARTESIAN_POINT ( 'NONE',  ( -100.1214030483830584, -286.5033629326264872, -231.8701936466242728 ) ) ;
#18755=CARTESIAN_POINT ( 'NONE',  ( -17.13707143614291439, -287.1224446259592469, -199.9919077277388908 ) ) ;
#18756=CARTESIAN_POINT ( 'NONE',  ( 21.80111255894472677, -294.8935796563231406, -223.6443142798336794 ) ) ;
#18757=CARTESIAN_POINT ( 'NONE',  ( -111.3874922928703199, -276.4393645415207743, -285.4762350049023212 ) ) ;
#18758=CARTESIAN_POINT ( 'NONE',  ( 23.50394265873821809, -276.5154624084473198, -317.5370524052583505 ) ) ;
#18759=CARTESIAN_POINT ( 'NONE',  ( -44.73141521653276698, -290.0392999602618147, -195.1114043686207538 ) ) ;
#18760=CARTESIAN_POINT ( 'NONE',  ( -101.8912199224298121, -279.1045746747556109, -228.2841715781802918 ) ) ;
#18761=CARTESIAN_POINT ( 'NONE',  ( -101.5691566137259372, -298.0197120064832461, -308.4980914793898705 ) ) ;
#18764=CARTESIAN_POINT ( 'NONE',  ( -22.34293603469879130, -284.9329319644132852, -198.3625115006764759 ) ) ;
#18765=CARTESIAN_POINT ( 'NONE',  ( -111.1345464317928560, -276.5808475524162304, -278.9089071990499633 ) ) ;
#18766=CARTESIAN_POINT ( 'NONE',  ( 37.70923014681355312, -279.5469251451431774, -269.9668807185926198 ) ) ;
#18768=CARTESIAN_POINT ( 'NONE',  ( -5.386818766784664092, -272.9448910365494498, -201.0675878931002956 ) ) ;
#18769=CARTESIAN_POINT ( 'NONE',  ( 34.12312648197760723, -295.3074112094442398, -288.3468432064793205 ) ) ;
#18770=CARTESIAN_POINT ( 'NONE',  ( -22.61202491430037398, -279.1566409615292628, -195.0440122638999583 ) ) ;
#18771=CARTESIAN_POINT ( 'NONE',  ( -67.38079478197782635, -296.3973111853301248, -337.1660434018394881 ) ) ;
#18772=CARTESIAN_POINT ( 'NONE',  ( -112.7150780685094418, -297.6984083220048092, -283.7807934834755201 ) ) ;
#18773=CARTESIAN_POINT ( 'NONE',  ( -105.4344203833179989, -272.5728162133851811, -243.8499151147408952 ) ) ;
#18774=CARTESIAN_POINT ( 'NONE',  ( -32.04067039278705664, -294.1191701816941304, -195.5357215786828533 ) ) ;
#18775=CARTESIAN_POINT ( 'NONE',  ( -105.4330856520122666, -285.1843091593478903, -234.2947129231015140 ) ) ;
#18776=CARTESIAN_POINT ( 'NONE',  ( 14.02801243071343507, -274.4803023513711082, -326.1232382290839382 ) ) ;
#18777=CARTESIAN_POINT ( 'NONE',  ( -14.95427692247031715, -288.6034048032812507, -344.0904954832176372 ) ) ;
#18778=CARTESIAN_POINT ( 'NONE',  ( 19.68919536766276579, -287.2584060330154330, -316.3054909557052952 ) ) ;
#18779=CARTESIAN_POINT ( 'NONE',  ( -47.44800378367437332, -289.9236734078226618, -195.9927533761947416 ) ) ;
#18781=CARTESIAN_POINT ( 'NONE',  ( -96.12512592106646991, -239.9971452530988358, -342.0757611934672582 ) ) ;
#18783=CARTESIAN_POINT ( 'NONE',  ( -50.76892163754745013, -288.7358408542963275, -342.2299572942357599 ) ) ;
#18785=CARTESIAN_POINT ( 'NONE',  ( -106.7876728478178592, -285.0730976505982994, -303.0731507119510866 ) ) ;
#18786=CARTESIAN_POINT ( 'NONE',  ( 21.13900441459611557, -291.9382306270628646, -220.6135005519547860 ) ) ;
#18787=CARTESIAN_POINT ( 'NONE',  ( -35.37728931260219412, -281.6765127216661995, -194.1734398434828393 ) ) ;
#18788=CARTESIAN_POINT ( 'NONE',  ( 12.65715879840846192, -282.0477568243366591, -212.4524625194193277 ) ) ;
#18789=CARTESIAN_POINT ( 'NONE',  ( -91.66646550385388537, -283.6873924885454699, -319.1428224308774588 ) ) ;
#18790=CARTESIAN_POINT ( 'NONE',  ( -7.931557987147630051, -278.6670339991420633, -339.3681074497190480 ) ) ;
#18791=CARTESIAN_POINT ( 'NONE',  ( -103.1155859552882106, -296.0293825643942682, -310.3960520175944566 ) ) ;
#18793=CARTESIAN_POINT ( 'NONE',  ( -91.94556639466898673, -289.2881740036900737, -219.4475847320395303 ) ) ;
#18794=CARTESIAN_POINT ( 'NONE',  ( -85.55952679142329487, -272.1628310167454288, -214.9564980983543308 ) ) ;
#18798=CARTESIAN_POINT ( 'NONE',  ( -111.6676273700015969, -286.5365823340550264, -265.3929911944862283 ) ) ;
#18799=CARTESIAN_POINT ( 'NONE',  ( 33.13794856051175941, -295.0199738230660955, -300.7295683472426617 ) ) ;
#18801=CARTESIAN_POINT ( 'NONE',  ( -34.83474700214905084, -283.6712813188154314, -343.4325059376524223 ) ) ;
#18802=CARTESIAN_POINT ( 'NONE',  ( -5.393661690203832570, -275.7007345470771611, -340.1618561865695938 ) ) ;
#18803=CARTESIAN_POINT ( 'NONE',  ( -111.1366832903113533, -291.4751518976114539, -248.7367510143157858 ) ) ;
#18804=CARTESIAN_POINT ( 'NONE',  ( -104.3287467996063498, -283.1575394208524585, -234.8505318502745354 ) ) ;
#18805=CARTESIAN_POINT ( 'NONE',  ( -79.58636089973413164, -291.8318217577649989, -205.9457621981620719 ) ) ;
#18806=CARTESIAN_POINT ( 'NONE',  ( -29.16654210983734785, -289.2789784196760934, -342.9231898805035144 ) ) ;
#18810=CARTESIAN_POINT ( 'NONE',  ( -107.3854158231707459, -264.5521555645648846, -305.4145383826947295 ) ) ;
#18811=CARTESIAN_POINT ( 'NONE',  ( -60.99817021723886512, -284.8737349944302082, -342.9633780162285461 ) ) ;
#18812=CARTESIAN_POINT ( 'NONE',  ( -4.771743288812454686, -283.9809262143061233, -202.8022627189028810 ) ) ;
#18814=CARTESIAN_POINT ( 'NONE',  ( 31.36480513695133610, -280.1311898739672301, -244.6489803408817636 ) ) ;
#18815=CARTESIAN_POINT ( 'NONE',  ( 36.04119379637801046, -275.5112173964161002, -293.6139709427035314 ) ) ;
#18816=CARTESIAN_POINT ( 'NONE',  ( -70.57688936365295262, -281.6130930180749488, -203.2988001691300326 ) ) ;
#18817=CARTESIAN_POINT ( 'NONE',  ( 47.02842677011826567, 10.69185302179798214, -329.9758182323871551 ) ) ;
#18818=CARTESIAN_POINT ( 'NONE',  ( 39.05232701943413076, -280.0857914278421958, -267.1007619881191317 ) ) ;
#18819=CARTESIAN_POINT ( 'NONE',  ( -103.6890943860418588, -283.0270031874921415, -236.1577544805183209 ) ) ;
#18820=CARTESIAN_POINT ( 'NONE',  ( -26.41416471961995072, -299.9473087259986528, -194.3712223735663542 ) ) ;
#18822=CARTESIAN_POINT ( 'NONE',  ( -42.38772121344757693, -295.6098550707359891, -343.2481958011119900 ) ) ;
#18825=CARTESIAN_POINT ( 'NONE',  ( -34.82372468284911093, -290.7692668114616481, -196.9111126810951191 ) ) ;
#18826=CARTESIAN_POINT ( 'NONE',  ( -14.61189703666436657, -277.4166366283656089, -343.8788947095050048 ) ) ;
#18827=CARTESIAN_POINT ( 'NONE',  ( 35.69883683584532008, -275.5682967614529844, -271.5849663936369325 ) ) ;
#18828=CARTESIAN_POINT ( 'NONE',  ( 1.052625872994708667, -273.4723967524362820, -203.9578800592401819 ) ) ;
#18830=CARTESIAN_POINT ( 'NONE',  ( -111.1113389439735215, -270.7292401098747519, -256.5566746695058100 ) ) ;
#18833=CARTESIAN_POINT ( 'NONE',  ( 28.43447001966500665, -283.0699600556689006, -302.8448902439720314 ) ) ;
#18834=CARTESIAN_POINT ( 'NONE',  ( 38.27215002563985280, -283.4140294380544560, -278.3888974233419162 ) ) ;
#18835=CARTESIAN_POINT ( 'NONE',  ( -109.7119693298962204, -284.0366421004114841, -260.0442965786539276 ) ) ;
#18836=CARTESIAN_POINT ( 'NONE',  ( -16.17065397512084957, -275.1738379208329093, -341.1128447602646929 ) ) ;
#18837=CARTESIAN_POINT ( 'NONE',  ( 14.80900492802579116, -284.1686893440596009, -323.2650374949166689 ) ) ;
#18838=CARTESIAN_POINT ( 'NONE',  ( -56.80172443905418334, -275.7873937937401934, -341.4916484449256586 ) ) ;
#18840=CARTESIAN_POINT ( 'NONE',  ( 33.54459041757150572, -276.8775938307750266, -289.0522893488450222 ) ) ;
#18842=CARTESIAN_POINT ( 'NONE',  ( -33.93268722918507052, -280.8968451076613633, -193.5982529248710478 ) ) ;
#18845=CARTESIAN_POINT ( 'NONE',  ( -75.50535936348644839, -287.4096260397911351, -204.8496377679980185 ) ) ;
#18846=CARTESIAN_POINT ( 'NONE',  ( -96.54509013646611493, -295.1488627145922692, -313.3657614661292996 ) ) ;
#18847=CARTESIAN_POINT ( 'NONE',  ( -112.4675391785426513, -289.6951900939840243, -286.7751697093871144 ) ) ;
#18848=CARTESIAN_POINT ( 'NONE',  ( 17.65845366658705018, -285.0924184874581897, -220.8148535762663016 ) ) ;
#18849=CARTESIAN_POINT ( 'NONE',  ( -10.51842168073719996, -284.9837870934871944, -201.8209416347469300 ) ) ;
#18850=CARTESIAN_POINT ( 'NONE',  ( -65.69470122671074819, -289.9160471312525260, -201.9801649349061847 ) ) ;
#18851=CARTESIAN_POINT ( 'NONE',  ( -104.9693623747481155, -286.1395522297913203, -241.7062207245768093 ) ) ;
#18852=CARTESIAN_POINT ( 'NONE',  ( 35.63964157812512212, -273.7745680289260690, -287.7000002103532097 ) ) ;
#18853=CARTESIAN_POINT ( 'NONE',  ( -51.99922893755491060, -284.2675810868524309, -195.5303123219319446 ) ) ;
#18854=CARTESIAN_POINT ( 'NONE',  ( -37.28144809524221159, -300.0530651647117679, -195.3603449120130335 ) ) ;
#18855=CARTESIAN_POINT ( 'NONE',  ( 36.97687297005811047, -285.4066402836695602, -259.0156515848358367 ) ) ;
#18856=CARTESIAN_POINT ( 'NONE',  ( -1.862551923666285747, -281.4757557258479324, -206.2936653162772132 ) ) ;
#18857=CARTESIAN_POINT ( 'NONE',  ( -71.06067032536718386, -291.4962940531041227, -337.5404263991663925 ) ) ;
#18861=CARTESIAN_POINT ( 'NONE',  ( -104.6633888595714410, -298.0207288525874105, -304.7852571985416148 ) ) ;
#18862=CARTESIAN_POINT ( 'NONE',  ( -60.32288788999900930, -277.7541595749368071, -198.9140230212935307 ) ) ;
#18863=CARTESIAN_POINT ( 'NONE',  ( -73.34897678022525724, -290.7841774309087555, -202.4666890109656379 ) ) ;
#18864=CARTESIAN_POINT ( 'NONE',  ( -73.21815732447144853, -295.9678506135770135, -205.8683258656144233 ) ) ;
#18865=CARTESIAN_POINT ( 'NONE',  ( 30.78544833183558183, -280.6036654770975360, -297.9280387326817845 ) ) ;
#18866=CARTESIAN_POINT ( 'NONE',  ( 21.84098360022365171, -273.0091043858556077, -225.1878949879414051 ) ) ;
#18867=CARTESIAN_POINT ( 'NONE',  ( 20.56114944821640833, -294.2333855278292845, -225.0803533602745858 ) ) ;
#18868=CARTESIAN_POINT ( 'NONE',  ( -85.28047601435906699, -298.1948066931273615, -330.5268031993605859 ) ) ;
#18869=CARTESIAN_POINT ( 'NONE',  ( -54.42098962299014175, -296.3164577819803753, -195.9903870379907005 ) ) ;
#18870=CARTESIAN_POINT ( 'NONE',  ( 38.48921935921545412, -291.8633059406286065, -275.9867490454769268 ) ) ;
#18872=CARTESIAN_POINT ( 'NONE',  ( -105.6533031316659503, -291.6124610939351669, -297.8638286415605307 ) ) ;
#18874=CARTESIAN_POINT ( 'NONE',  ( -69.09691759994316840, -292.4263627289237775, -204.4366782582059159 ) ) ;
#18876=CARTESIAN_POINT ( 'NONE',  ( -101.5304992912097788, -282.0451015658453571, -309.8352216879276853 ) ) ;
#18877=CARTESIAN_POINT ( 'NONE',  ( -14.84640119613110087, -292.3518903259908939, -200.9135728426330445 ) ) ;
#18878=CARTESIAN_POINT ( 'NONE',  ( 39.52916933180058834, -281.6184332394641956, -275.6608986983745808 ) ) ;
#18879=CARTESIAN_POINT ( 'NONE',  ( -81.55288412240864204, -283.3021188180685499, -333.4427560718260111 ) ) ;
#18881=CARTESIAN_POINT ( 'NONE',  ( -70.81484320899905072, -287.4945361477072652, -337.3049711775195192 ) ) ;
#18882=CARTESIAN_POINT ( 'NONE',  ( -1.444335248645383984, -278.9992547610586939, -203.0254888646603320 ) ) ;
#18884=CARTESIAN_POINT ( 'NONE',  ( 18.41062218692302110, -287.1945738057424933, -323.0220244139024430 ) ) ;
#18886=CARTESIAN_POINT ( 'NONE',  ( 34.42095219661052141, -294.9269111771769190, -253.0862142663106624 ) ) ;
#18887=CARTESIAN_POINT ( 'NONE',  ( 35.50640090569080343, -277.2694871423444170, -293.4210500843008163 ) ) ;
#18888=CARTESIAN_POINT ( 'NONE',  ( -93.10359974968768881, -278.8888814517983405, -223.1963870265717560 ) ) ;
#18889=CARTESIAN_POINT ( 'NONE',  ( 6.494488533721804124, -292.7966951989048994, -207.0571799684375378 ) ) ;
#18890=CARTESIAN_POINT ( 'NONE',  ( -64.75302457340447404, -281.4871486737209807, -340.7876528721564000 ) ) ;
#18891=CARTESIAN_POINT ( 'NONE',  ( 15.05219701163399826, -291.8722858071603810, -219.1192616871452685 ) ) ;
#18892=CARTESIAN_POINT ( 'NONE',  ( -111.6740538544493830, -294.4188869389090542, -280.7275134834287087 ) ) ;
#18895=CARTESIAN_POINT ( 'NONE',  ( 27.20950507223730241, -293.5268924276162466, -304.6909914870873308 ) ) ;
#18897=CARTESIAN_POINT ( 'NONE',  ( -102.0455923789670294, -293.6237833571632905, -301.4846348637937581 ) ) ;
#18898=CARTESIAN_POINT ( 'NONE',  ( -99.43051780650718285, -272.3524075826391027, -225.0055052814526846 ) ) ;
#18899=CARTESIAN_POINT ( 'NONE',  ( 5.505539833809690364, -278.7651994057787306, -207.8757636499558714 ) ) ;
#18900=CARTESIAN_POINT ( 'NONE',  ( 30.97387595866132415, -288.4212507545352651, -235.9186974031164254 ) ) ;
#18901=CARTESIAN_POINT ( 'NONE',  ( 27.02946414984780432, -287.8560809070183950, -304.8976562627448175 ) ) ;
#18902=CARTESIAN_POINT ( 'NONE',  ( -37.79477499226169357, -278.5780155439665009, -344.0656325535945257 ) ) ;
#18903=CARTESIAN_POINT ( 'NONE',  ( -108.4435728141672968, -294.2756057908904381, -293.2524164743741721 ) ) ;
#18904=CARTESIAN_POINT ( 'NONE',  ( -100.7767048361804427, -298.8309245426736993, -232.1303878486236272 ) ) ;
#18905=CARTESIAN_POINT ( 'NONE',  ( -110.0127458350879834, -277.4868049966538592, -259.7109375205692459 ) ) ;
#18906=EDGE_LOOP ( 'NONE', ( #50128, #66337 ) ) ;
#18907=CARTESIAN_POINT ( 'NONE',  ( -3.417821543773571946, -298.1327279901885277, -193.3841119163431586 ) ) ;
#18908=CARTESIAN_POINT ( 'NONE',  ( -102.8999741921116424, -291.9994475966411756, -305.7325986753883171 ) ) ;
#18909=CARTESIAN_POINT ( 'NONE',  ( 37.53530552031899958, -294.9736077720374965, -256.2234221980717166 ) ) ;
#18911=CARTESIAN_POINT ( 'NONE',  ( -96.84916500930633276, -291.7969625586382563, -227.8166296339977350 ) ) ;
#18913=CARTESIAN_POINT ( 'NONE',  ( -113.5019643645738796, -297.3378347527212782, -259.6390841796218751 ) ) ;
#18914=CARTESIAN_POINT ( 'NONE',  ( -98.05378919152518336, -288.0786964853737686, -315.7074932839720418 ) ) ;
#18915=CARTESIAN_POINT ( 'NONE',  ( -106.4961856110193850, -297.3197655250767752, -236.5468986506695899 ) ) ;
#18918=CARTESIAN_POINT ( 'NONE',  ( -29.03325661180904405, -290.4689228954406985, -346.2671623026141674 ) ) ;
#18919=CARTESIAN_POINT ( 'NONE',  ( 25.18497378105907814, -283.4090924074130839, -220.4570493818173702 ) ) ;
#18920=CARTESIAN_POINT ( 'NONE',  ( -73.27619907303937907, -287.5746980773051291, -204.7055472661805311 ) ) ;
#18921=CARTESIAN_POINT ( 'NONE',  ( 35.29463020705783549, -285.8242574056594663, -246.4732252129328458 ) ) ;
#18922=CARTESIAN_POINT ( 'NONE',  ( -66.50469390704590467, -271.6691758527842353, -201.4441518400082600 ) ) ;
#18923=CARTESIAN_POINT ( 'NONE',  ( -38.12150358451864918, -275.9624588189304859, -195.9251985070002604 ) ) ;
#18924=CARTESIAN_POINT ( 'NONE',  ( -102.3699398615240312, -289.1190763813115723, -234.0249009848026276 ) ) ;
#18925=CARTESIAN_POINT ( 'NONE',  ( -111.5785046087205075, -280.2193230442732101, -285.5645670620446595 ) ) ;
#18927=CARTESIAN_POINT ( 'NONE',  ( -14.30887690687654690, -280.3591643763424486, -201.0365515420852489 ) ) ;
#18928=CARTESIAN_POINT ( 'NONE',  ( -6.719158214782700256, -279.8136768529938081, -203.9685962304837119 ) ) ;
#18929=CARTESIAN_POINT ( 'NONE',  ( 14.68362212398608868, -277.4199162954646454, -326.7792892441633512 ) ) ;
#18930=CARTESIAN_POINT ( 'NONE',  ( 25.96119380767855844, -279.7741671649436057, -227.1320995106458156 ) ) ;
#18931=CARTESIAN_POINT ( 'NONE',  ( 101.5448465039121118, 115.7098217570894860, -280.1310368427940602 ) ) ;
#18932=CARTESIAN_POINT ( 'NONE',  ( 25.94377920860218723, -275.9179540940089623, -226.8893685182977151 ) ) ;
#18933=CARTESIAN_POINT ( 'NONE',  ( -97.28058710471766801, -274.7095762327166995, -223.1378442324793241 ) ) ;
#18934=CARTESIAN_POINT ( 'NONE',  ( -4.829096099716510437, -294.9805209788416391, -202.7746430608542312 ) ) ;
#18937=CARTESIAN_POINT ( 'NONE',  ( 13.34338273959105692, -287.8608674766525155, -217.3265000158627629 ) ) ;
#18938=CARTESIAN_POINT ( 'NONE',  ( 11.77807641742177225, -290.1408466456891801, -328.3371609959373245 ) ) ;
#18939=CARTESIAN_POINT ( 'NONE',  ( -108.2052430265821812, -290.1379391938208414, -252.3588819823835934 ) ) ;
#18940=AXIS2_PLACEMENT_3D ( 'NONE', #90959, #40773, #33703 ) ;
#18941=CARTESIAN_POINT ( 'NONE',  ( -35.14370753370436518, -285.5866794659120842, -193.4409260643512027 ) ) ;
#18943=CARTESIAN_POINT ( 'NONE',  ( -13.28766378687964789, -281.1344694934547306, -340.1852386514914315 ) ) ;
#18944=CARTESIAN_POINT ( 'NONE',  ( 6.594435684013265409, -290.3085974241698182, -330.2623200973995381 ) ) ;
#18945=CARTESIAN_POINT ( 'NONE',  ( -51.16677148893051452, -281.7118059978511155, -342.7980960525821388 ) ) ;
#18946=CARTESIAN_POINT ( 'NONE',  ( -72.37946481064477666, -280.8933190962096660, -205.7577239161643945 ) ) ;
#18947=CARTESIAN_POINT ( 'NONE',  ( 18.35939138315959340, -276.7161881296901242, -317.6408900450365422 ) ) ;
#18948=CARTESIAN_POINT ( 'NONE',  ( -97.14390731579817384, -289.9916753979920259, -222.4893649737437329 ) ) ;
#18950=CARTESIAN_POINT ( 'NONE',  ( -100.8687674336618016, -285.9272585173221159, -227.0413013179723976 ) ) ;
#18951=CARTESIAN_POINT ( 'NONE',  ( 12.03328035965071408, -287.2095133635745015, -211.2861942985843768 ) ) ;
#18952=CARTESIAN_POINT ( 'NONE',  ( 33.45506089537422412, -281.4833226953147118, -252.5109377799178390 ) ) ;
#18955=CARTESIAN_POINT ( 'NONE',  ( -105.3934700524614101, -291.9765227537372994, -303.7858825478775771 ) ) ;
#18956=CARTESIAN_POINT ( 'NONE',  ( -69.40113288861358853, -290.3239040214406259, -200.8811149789876254 ) ) ;
#18957=CARTESIAN_POINT ( 'NONE',  ( 22.47993516742575792, -274.0228657482211361, -228.0927434532131031 ) ) ;
#18959=CARTESIAN_POINT ( 'NONE',  ( -108.2842166799565859, -295.5212885965420355, -300.1717196851911922 ) ) ;
#18960=CARTESIAN_POINT ( 'NONE',  ( -63.02439339721960465, -290.1913948194979298, -201.2879175443906945 ) ) ;
#18961=CARTESIAN_POINT ( 'NONE',  ( -71.41701075110785268, -293.7483828484737387, -336.0780167449001965 ) ) ;
#18962=CARTESIAN_POINT ( 'NONE',  ( -45.39083524964373595, -290.3614852083207438, -343.3155004987569896 ) ) ;
#18964=CARTESIAN_POINT ( 'NONE',  ( -108.8665964327379214, -292.2592061424039684, -293.0958316240797217 ) ) ;
#18965=CARTESIAN_POINT ( 'NONE',  ( -19.78954960283480347, -290.2769892493946031, -197.2189484650397162 ) ) ;
#18966=CARTESIAN_POINT ( 'NONE',  ( -25.79620902928468951, -296.9053838787326072, -344.5188280773609222 ) ) ;
#18967=CARTESIAN_POINT ( 'NONE',  ( -4.499756205447580371, -287.4372382847431595, -204.9026183951946223 ) ) ;
#18968=CARTESIAN_POINT ( 'NONE',  ( 32.75132232384592612, -295.9046202709194517, -297.5087997985771153 ) ) ;
#18969=CARTESIAN_POINT ( 'NONE',  ( 36.86781725228782847, -277.3638169147595249, -257.1972860349069379 ) ) ;
#18970=CARTESIAN_POINT ( 'NONE',  ( 14.60259654582348965, -275.1355370406461702, -326.7342650939074247 ) ) ;
#18971=CARTESIAN_POINT ( 'NONE',  ( -73.19615735195343120, -296.7866442821683108, -202.3419951379497377 ) ) ;
#18972=CARTESIAN_POINT ( 'NONE',  ( -32.37463725636051493, -275.2286638592689201, -344.2582562883887931 ) ) ;
#18973=CARTESIAN_POINT ( 'NONE',  ( -67.87501289718414910, -277.7280919754755928, -202.4574011820792521 ) ) ;
#18974=CARTESIAN_POINT ( 'NONE',  ( -101.0701116958632610, -274.2546520269584107, -233.8470664991680508 ) ) ;
#18975=CARTESIAN_POINT ( 'NONE',  ( 0.9162446341252652449, -273.1268516302044986, -204.2026493507246414 ) ) ;
#18977=CARTESIAN_POINT ( 'NONE',  ( -108.0303867941109388, -298.2458317151121037, -249.9042243939786658 ) ) ;
#18979=CARTESIAN_POINT ( 'NONE',  ( -65.64460335955025982, -298.4751056735780139, -202.8959610797571713 ) ) ;
#18981=CARTESIAN_POINT ( 'NONE',  ( -8.878288440441002294, -286.7018021541762209, -340.1478584483220402 ) ) ;
#18982=CARTESIAN_POINT ( 'NONE',  ( -35.38819928235388090, -273.9106354040160909, -197.3747554587496040 ) ) ;
#18983=CARTESIAN_POINT ( 'NONE',  ( 19.62424641933716529, -288.2564058222681638, -322.1869436561482871 ) ) ;
#18984=CARTESIAN_POINT ( 'NONE',  ( -17.73380864816265401, -288.4726624259701566, -344.8008579280377717 ) ) ;
#18985=CARTESIAN_POINT ( 'NONE',  ( -62.32403971814561316, -299.7086724253267676, -199.2675914818975116 ) ) ;
#18986=CARTESIAN_POINT ( 'NONE',  ( 32.28213816380046097, -291.9115183161393361, -297.9354097082195381 ) ) ;
#18987=CARTESIAN_POINT ( 'NONE',  ( 30.58386087180263502, -280.2832315887928871, -234.3272300470326002 ) ) ;
#18989=CARTESIAN_POINT ( 'NONE',  ( -51.23241710295501861, -277.8745459040279115, -196.6064122313974281 ) ) ;
#18991=CARTESIAN_POINT ( 'NONE',  ( 10.36175281717805419, -287.1717352319661245, -326.2092279194358184 ) ) ;
#18993=CARTESIAN_POINT ( 'NONE',  ( -91.23628028588400696, -289.2856518755919524, -218.2039048864972415 ) ) ;
#18994=CARTESIAN_POINT ( 'NONE',  ( -99.87899047268398078, -274.6052608698339554, -231.3765688876021045 ) ) ;
#18995=CARTESIAN_POINT ( 'NONE',  ( 36.75539332297754669, -282.7421326655936582, -251.7002756421616425 ) ) ;
#18996=CARTESIAN_POINT ( 'NONE',  ( -81.97561402377259299, -295.4677244935770091, -209.5820480055150767 ) ) ;
#18997=CARTESIAN_POINT ( 'NONE',  ( -66.55957287216529039, -283.4457935327254745, -337.2724910204852904 ) ) ;
#18998=CARTESIAN_POINT ( 'NONE',  ( -8.758589379694553756, -275.8587566877072845, -202.4954172976708264 ) ) ;
#18999=CARTESIAN_POINT ( 'NONE',  ( 35.51574385217134733, -276.4426902996534068, -277.0240440181192980 ) ) ;
#19000=CARTESIAN_POINT ( 'NONE',  ( -14.01905113807645442, -284.7497394030690430, -341.6426351596688846 ) ) ;
#19001=CARTESIAN_POINT ( 'NONE',  ( -59.55627744073690621, -272.6780597559308603, -200.4456928389735708 ) ) ;
#19004=CARTESIAN_POINT ( 'NONE',  ( -11.05920414355691683, -294.5523030373764186, -342.7933069836394111 ) ) ;
#19005=CARTESIAN_POINT ( 'NONE',  ( -108.0993679551943956, -286.8427680437682170, -246.4251853724435648 ) ) ;
#19007=CARTESIAN_POINT ( 'NONE',  ( 25.18497378105905682, -273.6952119285918457, -320.2651865833026363 ) ) ;
#19008=CARTESIAN_POINT ( 'NONE',  ( -68.95829563863719613, -276.6545694870480361, -340.4079838042694632 ) ) ;
#19009=CARTESIAN_POINT ( 'NONE',  ( -110.8555608138664752, -289.2064009549977754, -250.2579103794683135 ) ) ;
#19010=CARTESIAN_POINT ( 'NONE',  ( -74.12624196631004736, -285.0702095508625575, -334.2753906971367996 ) ) ;
#19012=CARTESIAN_POINT ( 'NONE',  ( -8.320972237583498909, -278.4270535124706498, -338.4613497847494159 ) ) ;
#19013=CARTESIAN_POINT ( 'NONE',  ( -73.97739404131314700, -284.9538915480133596, -337.4755898145663764 ) ) ;
#19014=CARTESIAN_POINT ( 'NONE',  ( -21.31638399556991459, -281.6370667660092408, -342.0396619241350891 ) ) ;
#19015=CARTESIAN_POINT ( 'NONE',  ( -2.234859526198311297, -282.5169013349871534, -204.0705372737294567 ) ) ;
#19016=CARTESIAN_POINT ( 'NONE',  ( 28.50144580648328230, -275.1965741415396565, -230.3382679360367149 ) ) ;
#19017=CARTESIAN_POINT ( 'NONE',  ( -104.9765986667826070, -277.9092091799133186, -307.1649289828673659 ) ) ;
#19018=CARTESIAN_POINT ( 'NONE',  ( -36.96416287557057245, -296.9675092877473048, -344.8128343504163240 ) ) ;
#19020=CARTESIAN_POINT ( 'NONE',  ( -109.6285296886695733, -294.4014580894347546, -293.0964298822452747 ) ) ;
#19021=CARTESIAN_POINT ( 'NONE',  ( 17.47725363303493751, -275.7491181336600334, -318.6797906538209872 ) ) ;
#19022=CARTESIAN_POINT ( 'NONE',  ( -113.9451976302604379, -273.7928955659290295, -267.5237491005502761 ) ) ;
#19023=CARTESIAN_POINT ( 'NONE',  ( 36.56304859358461101, -289.2490275679292040, -265.4980928583517539 ) ) ;
#19024=CARTESIAN_POINT ( 'NONE',  ( -85.93873637189760473, -297.2317184728580060, -329.1916867306165386 ) ) ;
#19025=CARTESIAN_POINT ( 'NONE',  ( 33.05774922560197382, -295.1453579721232927, -300.6932587163273638 ) ) ;
#19026=CARTESIAN_POINT ( 'NONE',  ( -103.2459557649118551, -292.0794411352630959, -305.9202800335608003 ) ) ;
#19027=CARTESIAN_POINT ( 'NONE',  ( -30.05924010357734133, -278.1442228727949555, -195.8313521715718935 ) ) ;
#19028=CARTESIAN_POINT ( 'NONE',  ( -109.3720579153232961, -280.7161279424268514, -251.5242396855583706 ) ) ;
#19029=CARTESIAN_POINT ( 'NONE',  ( -111.8253227037627511, -294.6177698717550015, -271.4604521233549121 ) ) ;
#19030=CARTESIAN_POINT ( 'NONE',  ( -0.9476217701010717365, -284.4347738489031485, -336.8271290643297107 ) ) ;
#19031=CARTESIAN_POINT ( 'NONE',  ( 35.86220529250802258, -286.4096721109496571, -265.5801862427985043 ) ) ;
#19032=CARTESIAN_POINT ( 'NONE',  ( 46.88546938567958478, 11.31389355509462291, -331.4406996308803741 ) ) ;
#19034=CARTESIAN_POINT ( 'NONE',  ( -57.39611940224994413, -285.4529398884592410, -200.0951886219402525 ) ) ;
#19036=CARTESIAN_POINT ( 'NONE',  ( 17.61440780927308936, -283.3688226009854247, -323.9283089932884536 ) ) ;
#19037=CARTESIAN_POINT ( 'NONE',  ( -48.88296166321605085, -274.2345039754250706, -198.2066231337833528 ) ) ;
#19038=CARTESIAN_POINT ( 'NONE',  ( -15.51184499926307581, -285.1233564870236137, -196.8794037206927783 ) ) ;
#19039=CARTESIAN_POINT ( 'NONE',  ( -38.17939962249425179, -280.9831412569245686, -193.6009820160768982 ) ) ;
#19041=CARTESIAN_POINT ( 'NONE',  ( -67.10999394045602173, -281.1890335110183514, -200.1004857822151735 ) ) ;
#19042=CARTESIAN_POINT ( 'NONE',  ( 29.26616279052587899, -281.3834569720291370, -231.7717815167536912 ) ) ;
#19043=CARTESIAN_POINT ( 'NONE',  ( 7.399455738971487229, -279.9094976428775681, -326.5171145203363494 ) ) ;
#19044=CARTESIAN_POINT ( 'NONE',  ( 190.6848901948926027, 270.9012093486809363, -139.6392467641786368 ) ) ;
#19046=CARTESIAN_POINT ( 'NONE',  ( 22.12322928847072490, -276.9287847433913043, -224.9093112442553490 ) ) ;
#19047=CARTESIAN_POINT ( 'NONE',  ( 44.58079383892317793, 12.73659974197433620, -331.8102939384928050 ) ) ;
#19048=CARTESIAN_POINT ( 'NONE',  ( 18.82626069481717224, -280.2583195277787240, -319.5241832013510361 ) ) ;
#19049=CARTESIAN_POINT ( 'NONE',  ( -36.41356295141496702, -293.8237733903442859, -194.3672561163407693 ) ) ;
#19050=CARTESIAN_POINT ( 'NONE',  ( -20.83320936382524380, -294.1833337229817289, -341.6267926717862338 ) ) ;
#19051=CARTESIAN_POINT ( 'NONE',  ( -44.88476794646827983, -291.4668766204152348, -193.7404312595681404 ) ) ;
#19053=CARTESIAN_POINT ( 'NONE',  ( -83.84112659353174024, -294.2509448288038811, -331.0612449030070366 ) ) ;
#19054=CARTESIAN_POINT ( 'NONE',  ( 34.16875774102882701, -285.7132766600460059, -252.0701301054242265 ) ) ;
#19055=CARTESIAN_POINT ( 'NONE',  ( 29.51715895196011985, -295.8432727049249138, -302.7405321901514412 ) ) ;
#19056=CARTESIAN_POINT ( 'NONE',  ( 27.45742738705570574, -286.7077717641705021, -305.1438205458529751 ) ) ;
#19057=CARTESIAN_POINT ( 'NONE',  ( -105.0584267521073087, -286.2496327910332639, -241.6699811892725052 ) ) ;
#19059=CARTESIAN_POINT ( 'NONE',  ( -44.88588853948748891, -292.9002446658929557, -193.9152591176198825 ) ) ;
#19060=CARTESIAN_POINT ( 'NONE',  ( -29.43176443758198246, -283.4417474349663735, -343.0437602525310581 ) ) ;
#19061=CARTESIAN_POINT ( 'NONE',  ( -113.9407591959636079, -295.3567574941754970, -269.5911391662599499 ) ) ;
#19062=CARTESIAN_POINT ( 'NONE',  ( -94.59782229122845365, -292.0515202943333293, -219.1176277080542150 ) ) ;
#19063=CARTESIAN_POINT ( 'NONE',  ( -13.89118181700644428, -292.8406952314584828, -197.0276341407994209 ) ) ;
#19064=CARTESIAN_POINT ( 'NONE',  ( 32.31425617400080341, -288.0103094660927354, -292.3707967870726065 ) ) ;
#19067=CARTESIAN_POINT ( 'NONE',  ( -100.5839457998255995, -297.8538944069742911, -312.1779388397400226 ) ) ;
#19068=CARTESIAN_POINT ( 'NONE',  ( -20.62698905467090071, -296.9421269185311303, -193.8579100128171149 ) ) ;
#19069=CARTESIAN_POINT ( 'NONE',  ( -1.841558484049782729, -279.5935557865460055, -206.3052955172217651 ) ) ;
#19072=CARTESIAN_POINT ( 'NONE',  ( 38.86408800217596138, -274.9272246995406590, -259.7684432184076400 ) ) ;
#19073=CARTESIAN_POINT ( 'NONE',  ( -95.82762422071574804, -295.6570911407147833, -225.5063748874037231 ) ) ;
#19074=CARTESIAN_POINT ( 'NONE',  ( -74.61328858115132334, -279.4141855127528515, -334.5615399034859365 ) ) ;
#19075=CARTESIAN_POINT ( 'NONE',  ( 35.84738177226173406, -273.5296548867451634, -257.8667889600991430 ) ) ;
#19076=CARTESIAN_POINT ( 'NONE',  ( -88.76917945675440080, -296.9986580170072443, -322.7999311888759735 ) ) ;
#19077=CARTESIAN_POINT ( 'NONE',  ( -107.7601042620882339, -297.9002866353736181, -249.9779280146009626 ) ) ;
#19079=CARTESIAN_POINT ( 'NONE',  ( -110.8151805956194806, -297.8965663403694180, -290.5623081628882574 ) ) ;
#19080=CARTESIAN_POINT ( 'NONE',  ( -51.43137961469841457, -295.8723580471684045, -196.4737386689759546 ) ) ;
#19081=CARTESIAN_POINT ( 'NONE',  ( -72.68349467631576033, -292.2227669743808747, -206.3132154034420580 ) ) ;
#19082=CARTESIAN_POINT ( 'NONE',  ( -86.30767457985406566, -289.9318046556179524, -215.3588743740152154 ) ) ;
#19083=DIRECTION ( 'NONE',  ( -1.000000000000000000, -0.000000000000000000, -0.000000000000000000 ) ) ;
#19084=CARTESIAN_POINT ( 'NONE',  ( 35.66956938950480804, -275.7368775982211559, -245.9263411066081346 ) ) ;
#19085=CARTESIAN_POINT ( 'NONE',  ( -71.90960281324012726, -273.7487489490164307, -206.0081361520411747 ) ) ;
#19086=CARTESIAN_POINT ( 'NONE',  ( -3.159272911374352955, -282.4812220372008937, -203.1904080733705769 ) ) ;
#19088=CARTESIAN_POINT ( 'NONE',  ( 21.22165363788893444, -280.9041633259438413, -319.5915137754943203 ) ) ;
#19089=CARTESIAN_POINT ( 'NONE',  ( -93.26557235102262666, -277.1784327708272144, -323.2185305411105674 ) ) ;
#19090=CARTESIAN_POINT ( 'NONE',  ( -109.5789386915224526, -283.9029449644849024, -258.6894596859793864 ) ) ;
#19091=CARTESIAN_POINT ( 'NONE',  ( 3.527015550632476515, -280.5041807362050008, -333.5080933350487271 ) ) ;
#19093=CARTESIAN_POINT ( 'NONE',  ( -91.54435054112427395, -271.8357250074435569, -220.5685046757476186 ) ) ;
#19094=CARTESIAN_POINT ( 'NONE',  ( -37.76180476151213128, -279.0575998057332754, -345.3725049901557895 ) ) ;
#19097=CARTESIAN_POINT ( 'NONE',  ( -113.5417001291471024, -270.9522813053617369, -270.3407899428912629 ) ) ;
#19098=CARTESIAN_POINT ( 'NONE',  ( -112.2200814915740068, -280.6438772235991905, -263.2141941308548780 ) ) ;
#19099=CARTESIAN_POINT ( 'NONE',  ( -40.84350783984969979, -272.0080689485911876, -195.3918459206030604 ) ) ;
#19100=DIRECTION ( 'NONE',  ( -1.000000000000000000, -0.000000000000000000, -0.000000000000000000 ) ) ;
#19101=CARTESIAN_POINT ( 'NONE',  ( -107.6968004657215232, -286.8299134348403641, -242.6601490968003816 ) ) ;
#19102=CARTESIAN_POINT ( 'NONE',  ( -9.696358412319998621, -286.6908782887689995, -340.0937875371106429 ) ) ;
#19104=CARTESIAN_POINT ( 'NONE',  ( 33.12712816227236345, -292.6176458556732314, -290.9312367272567030 ) ) ;
#19105=CARTESIAN_POINT ( 'NONE',  ( 24.57721647626301831, -285.1319718354183692, -229.3178761208892524 ) ) ;
#19106=CARTESIAN_POINT ( 'NONE',  ( 202.9738562182569694, 296.4636489450776367, -53.99999999999997868 ) ) ;
#19107=CARTESIAN_POINT ( 'NONE',  ( -111.7929898901849981, -294.4303608837819866, -279.8338554059012608 ) ) ;
#19108=CARTESIAN_POINT ( 'NONE',  ( -0.03809412471642474596, -285.0190603887202769, -203.7793299268059570 ) ) ;
#19109=CARTESIAN_POINT ( 'NONE',  ( 34.53495670390901040, -282.9338591087963550, -253.6223420304083334 ) ) ;
#19110=CARTESIAN_POINT ( 'NONE',  ( 38.62850208667887841, -279.7509763932390570, -267.1232116835210491 ) ) ;
#19111=CARTESIAN_POINT ( 'NONE',  ( -88.66106809430590374, -289.7972933910598385, -322.2776131603669114 ) ) ;
#19112=CARTESIAN_POINT ( 'NONE',  ( -107.0083868980533026, -280.2917782631946579, -246.4995038274308286 ) ) ;
#19113=CARTESIAN_POINT ( 'NONE',  ( -11.69610293760054276, -281.1975261912533597, -201.7881685346277436 ) ) ;
#19114=CARTESIAN_POINT ( 'NONE',  ( 36.50164532655497851, -289.7239724984143550, -285.3800106942805428 ) ) ;
#19116=CARTESIAN_POINT ( 'NONE',  ( -113.0682893601508709, -272.7301230832840133, -256.1307079426312612 ) ) ;
#19117=CARTESIAN_POINT ( 'NONE',  ( -111.8898848917655755, -292.5927436484923874, -265.6565254940458658 ) ) ;
#19119=CARTESIAN_POINT ( 'NONE',  ( -99.86837403722181250, -292.4090924074130839, -320.2651865833026363 ) ) ;
#19121=CARTESIAN_POINT ( 'NONE',  ( 35.51468649724040461, -273.3149533264262345, -251.8685422326711887 ) ) ;
#19122=DIRECTION ( 'NONE',  ( 1.000000000000000000, 0.000000000000000000, 0.000000000000000000 ) ) ;
#19123=CARTESIAN_POINT ( 'NONE',  ( -103.9140130235631432, -294.4651158269297184, -307.5441959380592039 ) ) ;
#19124=CARTESIAN_POINT ( 'NONE',  ( -99.94629275890376618, -296.5787989552235331, -232.5977301564361142 ) ) ;
#19125=CARTESIAN_POINT ( 'NONE',  ( -7.924091673659301449, -290.1798445040051888, -337.9827716403593172 ) ) ;
#19126=CARTESIAN_POINT ( 'NONE',  ( -8.073175706643860750, -284.4235629146169231, -338.3414643579641847 ) ) ;
#19127=CARTESIAN_POINT ( 'NONE',  ( -53.28423573993921281, -293.2769756701276265, -195.5779116826343227 ) ) ;
#19128=CARTESIAN_POINT ( 'NONE',  ( -65.25141332893073809, -290.7244247455753339, -341.6515393523510511 ) ) ;
#19129=CARTESIAN_POINT ( 'NONE',  ( -97.38191157747579041, -287.1663516298240211, -225.4147759636723549 ) ) ;
#19130=CARTESIAN_POINT ( 'NONE',  ( -97.69821886276980649, -279.3586402124670371, -222.5480376512654175 ) ) ;
#19131=CARTESIAN_POINT ( 'NONE',  ( -101.0881710472737041, -295.1738866049096828, -229.7938695864031899 ) ) ;
#19132=CARTESIAN_POINT ( 'NONE',  ( 22.52192514762148789, -282.0350669651697331, -318.8106966827294855 ) ) ;
#19133=CARTESIAN_POINT ( 'NONE',  ( 16.32361754381321717, -276.6842517230317640, -218.9944411785646423 ) ) ;
#19134=CARTESIAN_POINT ( 'NONE',  ( -82.13390479932378696, -275.9090924074130271, -214.2458315076590907 ) ) ;
#19135=CARTESIAN_POINT ( 'NONE',  ( -109.4977049187817499, -276.3945724307605474, -293.6346733324220963 ) ) ;
#19137=CARTESIAN_POINT ( 'NONE',  ( 21.38217294224192599, -280.4506154646063578, -226.8717355002970351 ) ) ;
#19138=CARTESIAN_POINT ( 'NONE',  ( -108.2829020371179212, -279.3882418821172564, -299.2636194198420867 ) ) ;
#19139=CARTESIAN_POINT ( 'NONE',  ( -35.14292900344018733, -285.1378472560713817, -193.6148041650766345 ) ) ;
#19140=CARTESIAN_POINT ( 'NONE',  ( -52.60027132107033054, -293.6142978870089451, -197.8850852416966291 ) ) ;
#19141=CARTESIAN_POINT ( 'NONE',  ( 31.14530127559968165, -277.5870547306427056, -303.8875214355168737 ) ) ;
#19142=CARTESIAN_POINT ( 'NONE',  ( 26.50970416140871322, -276.3095048748384102, -228.2149859799214369 ) ) ;
#19144=CARTESIAN_POINT ( 'NONE',  ( 35.37841573153354346, -275.2939439364304803, -263.4228568230018368 ) ) ;
#19145=CARTESIAN_POINT ( 'NONE',  ( -110.0750188786464321, -298.3250803534549505, -288.0188526371112516 ) ) ;
#19146=CARTESIAN_POINT ( 'NONE',  ( -110.9929811818575871, -282.7234030662491477, -257.0408724347454950 ) ) ;
#19147=CARTESIAN_POINT ( 'NONE',  ( 24.79989469958890780, -292.6155192340553413, -224.9280189923490241 ) ) ;
#19148=CARTESIAN_POINT ( 'NONE',  ( -40.28721907734122709, -290.6886905126430065, -346.5171157729111542 ) ) ;
#19149=CARTESIAN_POINT ( 'NONE',  ( -7.130349273065858640, -291.3784279388920595, -203.5666544844541477 ) ) ;
#19151=CARTESIAN_POINT ( 'NONE',  ( -2.309683589954180771, -291.0812126288142281, -202.4394264261509591 ) ) ;
#19152=CARTESIAN_POINT ( 'NONE',  ( -34.85231234756710705, -291.7510008970354534, -197.3824194786699593 ) ) ;
#19154=CARTESIAN_POINT ( 'NONE',  ( 37.80815125157658230, -288.8238973310369033, -285.6579264225256338 ) ) ;
#19156=CARTESIAN_POINT ( 'NONE',  ( -88.40988614964473413, -294.6681969542845536, -327.6471383155461581 ) ) ;
#19157=CARTESIAN_POINT ( 'NONE',  ( -107.8360113200843671, -285.5972411640034352, -239.5055597734092316 ) ) ;
#19158=CARTESIAN_POINT ( 'NONE',  ( 32.69102699790111188, -287.4753688959346505, -238.2771976502217228 ) ) ;
#19159=CARTESIAN_POINT ( 'NONE',  ( -21.37946038499688228, -283.1751761666347988, -341.6682823668233482 ) ) ;
#19160=CARTESIAN_POINT ( 'NONE',  ( 179.8324430359451469, 254.2804809356018438, -166.6962587909805507 ) ) ;
#19161=CARTESIAN_POINT ( 'NONE',  ( 195.8903196521388850, 285.0434368066629531, -111.3771662356307246 ) ) ;
#19162=CARTESIAN_POINT ( 'NONE',  ( 195.5810153702553578, 282.4170139924178784, -110.2874269805470533 ) ) ;
#19163=CARTESIAN_POINT ( 'NONE',  ( 19.98840512737379171, -274.1089791189192511, -224.8893273668976462 ) ) ;
#19164=CARTESIAN_POINT ( 'NONE',  ( 16.74998684707813013, -275.1794960946866695, -319.8602924183693403 ) ) ;
#19165=CARTESIAN_POINT ( 'NONE',  ( -113.3277794448817417, -296.2119018351638147, -258.2094495888708252 ) ) ;
#19166=CARTESIAN_POINT ( 'NONE',  ( -68.96539051565628142, -196.7406117984471052, -357.3712819849171751 ) ) ;
#19167=CARTESIAN_POINT ( 'NONE',  ( -1.712334662834919641, -275.2748333539560690, -338.0652285700219863 ) ) ;
#19168=CARTESIAN_POINT ( 'NONE',  ( -34.44277719179873287, -299.9492309039443967, -196.1249797147749518 ) ) ;
#19169=CARTESIAN_POINT ( 'NONE',  ( -40.44279298285383817, -298.9554434094916360, -193.6071081001820744 ) ) ;
#19170=CARTESIAN_POINT ( 'NONE',  ( 28.86307556313219891, -287.6275786598560558, -239.4594009245641644 ) ) ;
#19171=CARTESIAN_POINT ( 'NONE',  ( -41.92568613099764008, -295.9112267315418308, -347.1150699620685032 ) ) ;
#19172=CARTESIAN_POINT ( 'NONE',  ( -62.83057623854973173, -298.2213672155115773, -197.7674261231517505 ) ) ;
#19173=CARTESIAN_POINT ( 'NONE',  ( 24.42838960059447473, -294.2573577986904638, -309.3592381204121011 ) ) ;
#19175=CARTESIAN_POINT ( 'NONE',  ( 38.11471748469551812, -277.4104489510829126, -265.5074445544746595 ) ) ;
#19176=CARTESIAN_POINT ( 'NONE',  ( -67.33268488774348270, -279.1768894789483397, -199.5086816342627003 ) ) ;
#19177=CARTESIAN_POINT ( 'NONE',  ( -85.25014032811193943, -278.6741182138933368, -325.8195270661732934 ) ) ;
#19178=CARTESIAN_POINT ( 'NONE',  ( 38.37272345668768025, -277.3937367117095505, -276.7876312898428637 ) ) ;
#19179=CARTESIAN_POINT ( 'NONE',  ( -59.21224747668785682, -275.3539658206864260, -342.4727395087656419 ) ) ;
#19180=CARTESIAN_POINT ( 'NONE',  ( -94.53625257169122165, -297.8455756013553923, -224.8344682116025410 ) ) ;
#19181=CARTESIAN_POINT ( 'NONE',  ( -50.59499754121058857, -293.7994611848385489, -342.7470629117134990 ) ) ;
#19183=CARTESIAN_POINT ( 'NONE',  ( -67.34424839344553959, -280.1614247869131873, -199.5135774400097830 ) ) ;
#19184=CARTESIAN_POINT ( 'NONE',  ( -108.6072184209689055, -278.9281931386223619, -254.4853564134882333 ) ) ;
#19185=CARTESIAN_POINT ( 'NONE',  ( 36.30511850056931422, -286.4989011540779416, -291.1321638049303147 ) ) ;
#19186=CARTESIAN_POINT ( 'NONE',  ( -30.71290953486229824, -300.1351034432233860, -195.1921889355453743 ) ) ;
#19189=CARTESIAN_POINT ( 'NONE',  ( -42.68589332596516783, -288.3183194308615498, -343.3778625224693997 ) ) ;
#19190=CARTESIAN_POINT ( 'NONE',  ( -7.571567205648026544, -278.6876960848901490, -202.5850723548841472 ) ) ;
#19191=CARTESIAN_POINT ( 'NONE',  ( -99.95964648073017145, -277.6568281901861610, -231.6068914038433206 ) ) ;
#19192=CARTESIAN_POINT ( 'NONE',  ( -32.06760748982689080, -281.0649392113111844, -344.6140515634363055 ) ) ;
#19193=CARTESIAN_POINT ( 'NONE',  ( -106.2146468188840487, -286.9421581721882148, -240.5416067929351698 ) ) ;
#19194=CARTESIAN_POINT ( 'NONE',  ( -97.96820939095927372, -279.1847433690685421, -311.7320846099459004 ) ) ;
#19196=CARTESIAN_POINT ( 'NONE',  ( -35.04778466501801404, -294.0810897511464646, -195.3833934152537211 ) ) ;
#19197=CARTESIAN_POINT ( 'NONE',  ( -77.30133824385073638, -275.8196281508062384, -335.0535451644575460 ) ) ;
#19198=CARTESIAN_POINT ( 'NONE',  ( -13.74465827841398102, -277.3891975232490950, -339.6030040671423080 ) ) ;
#19199=CARTESIAN_POINT ( 'NONE',  ( -89.15549691237981733, -285.7786127769256268, -324.8875706930659248 ) ) ;
#19201=CARTESIAN_POINT ( 'NONE',  ( -96.15354890874544935, -291.8239821709321404, -317.8207460599227261 ) ) ;
#19202=CARTESIAN_POINT ( 'NONE',  ( -95.93821868842539402, -293.9081572155508297, -317.1941802727007484 ) ) ;
#19204=CARTESIAN_POINT ( 'NONE',  ( 31.28218055757993454, -286.3035850472850257, -235.7934767607450226 ) ) ;
#19206=CARTESIAN_POINT ( 'NONE',  ( 5.671946108636324979, -275.1408140073654067, -330.0148047846920463 ) ) ;
#19207=CARTESIAN_POINT ( 'NONE',  ( 32.69768401439767302, -292.0154469445254222, -295.1187568085193789 ) ) ;
#19210=CARTESIAN_POINT ( 'NONE',  ( -44.80974917579993644, -290.4392675593994113, -194.3683274290261238 ) ) ;
#19211=CARTESIAN_POINT ( 'NONE',  ( -86.27163083601209337, -286.9602894620695110, -215.0451526915797160 ) ) ;
#19212=CARTESIAN_POINT ( 'NONE',  ( 35.80281138171877586, -286.0540058276777700, -290.9965100657445305 ) ) ;
#19213=CARTESIAN_POINT ( 'NONE',  ( -110.8988318193390796, -286.0058719838534103, -268.1878041858792585 ) ) ;
#19214=EDGE_CURVE ( 'NONE', #6475, #62648, #26070, .T. ) ;
#19216=CARTESIAN_POINT ( 'NONE',  ( -73.64462034686829384, -286.3599454160650453, -206.8273026964639598 ) ) ;
#19217=CARTESIAN_POINT ( 'NONE',  ( 37.58773696906638406, -295.4237301880644395, -261.8853295629847366 ) ) ;
#19218=CARTESIAN_POINT ( 'NONE',  ( -4.640606255320009588, -274.7046195760476053, -338.4925409304452160 ) ) ;
#19219=CARTESIAN_POINT ( 'NONE',  ( 14.87195484190964656, -276.6736462525976208, -326.9976038943935350 ) ) ;
#19220=CARTESIAN_POINT ( 'NONE',  ( -53.06533541039279100, -289.9320876350648746, -196.4017464581970103 ) ) ;
#19221=CARTESIAN_POINT ( 'NONE',  ( -99.42786816593280719, -279.1572650174151136, -224.7942965060165363 ) ) ;
#19222=CARTESIAN_POINT ( 'NONE',  ( -71.66517040781522496, -297.4878114800368394, -336.6607546392650647 ) ) ;
#19225=CARTESIAN_POINT ( 'NONE',  ( -30.46859702267936143, -284.8255638981279958, -197.1389164006562851 ) ) ;
#19226=CARTESIAN_POINT ( 'NONE',  ( -97.90694129153108349, -276.1020812294920006, -313.3100845624825297 ) ) ;
#19227=CARTESIAN_POINT ( 'NONE',  ( 12.33647257618995674, -280.3607973171270373, -326.6181222355833143 ) ) ;
#19229=CARTESIAN_POINT ( 'NONE',  ( 35.07813996601782236, -273.7247329064165342, -246.1512484178971647 ) ) ;
#19230=CARTESIAN_POINT ( 'NONE',  ( -80.88673780970184168, -277.0098056950945988, -329.0784268544667270 ) ) ;
#19231=CARTESIAN_POINT ( 'NONE',  ( -7.691753305845443478, -296.1764699141970709, -337.8402871408548549 ) ) ;
#19233=CARTESIAN_POINT ( 'NONE',  ( 38.96906939831934835, -280.5746744134050346, -278.4994459607108865 ) ) ;
#19234=CARTESIAN_POINT ( 'NONE',  ( -20.78335903422243902, -295.7757426783928167, -341.7522306533316510 ) ) ;
#19235=CARTESIAN_POINT ( 'NONE',  ( -36.91721156693651551, -299.3725293809989694, -193.8541723928366309 ) ) ;
#19236=CARTESIAN_POINT ( 'NONE',  ( -110.2095571528937796, -272.2907884077905578, -264.9076476289289985 ) ) ;
#19237=CARTESIAN_POINT ( 'NONE',  ( -82.96532920742994577, -293.4285347675631215, -210.7682030704291094 ) ) ;
#19238=CARTESIAN_POINT ( 'NONE',  ( -35.15036386621238051, -286.2456001408052657, -193.3791623395837860 ) ) ;
#19239=CARTESIAN_POINT ( 'NONE',  ( 37.90785305008348871, -273.8094307723012548, -279.6208324128426170 ) ) ;
#19240=CARTESIAN_POINT ( 'NONE',  ( 28.90266363740056832, -287.8968621647022701, -309.6126692104884910 ) ) ;
#19241=CARTESIAN_POINT ( 'NONE',  ( -32.88954751117633180, -282.0884243912386182, -195.8492052368922884 ) ) ;
#19242=CARTESIAN_POINT ( 'NONE',  ( 34.80128781790409676, -286.4414312600176231, -257.4733000395002023 ) ) ;
#19243=CARTESIAN_POINT ( 'NONE',  ( -52.94763135209608151, -289.8520940826414858, -196.9496342952077157 ) ) ;
#19245=CARTESIAN_POINT ( 'NONE',  ( 164.1991770243031681, 231.0496910105122765, -188.4318802409405009 ) ) ;
#19246=CARTESIAN_POINT ( 'NONE',  ( 32.73076934925363446, -286.7858086738262386, -249.6327390865224345 ) ) ;
#19248=CARTESIAN_POINT ( 'NONE',  ( 0.7620111289098248086, -283.4981740433552773, -337.0165884279342663 ) ) ;
#19249=CARTESIAN_POINT ( 'NONE',  ( -111.0029971093512557, -289.8827438656514914, -248.7547869612925240 ) ) ;
#19250=CARTESIAN_POINT ( 'NONE',  ( 0.9541017032971741418, -282.1539631844422047, -204.4233466335672347 ) ) ;
#19251=CARTESIAN_POINT ( 'NONE',  ( 32.71461710192765082, -282.4726592047770168, -239.6135865750992195 ) ) ;
#19252=CARTESIAN_POINT ( 'NONE',  ( 34.70321745139083447, -281.5407355279730268, -282.1309886479731972 ) ) ;
#19253=CARTESIAN_POINT ( 'NONE',  ( 35.53583224254434469, -277.7804538051685199, -288.1315569825152352 ) ) ;
#19254=CARTESIAN_POINT ( 'NONE',  ( 13.39582739010140955, -294.3653761964523028, -328.3516132997970089 ) ) ;
#19255=CARTESIAN_POINT ( 'NONE',  ( -95.55821391285505229, -289.2182366478500626, -223.6216074237341047 ) ) ;
#19256=CARTESIAN_POINT ( 'NONE',  ( -94.07557479271419254, -272.0033672433459628, -223.7754103272211808 ) ) ;
#19259=CARTESIAN_POINT ( 'NONE',  ( -97.06267273757688940, -285.8610062081989440, -314.7989355585051499 ) ) ;
#19260=CARTESIAN_POINT ( 'NONE',  ( 37.16300026672992374, -294.8607809645405382, -288.5969262331369691 ) ) ;
#19261=CARTESIAN_POINT ( 'NONE',  ( 17.68705264205629035, -282.8891997407130248, -318.4831403524349298 ) ) ;
#19262=CARTESIAN_POINT ( 'NONE',  ( 25.86630329801068129, -275.1888213164584727, -314.0141914818792088 ) ) ;
#19263=CARTESIAN_POINT ( 'NONE',  ( -110.3367714222608953, -291.5102982578577553, -246.0069840434583455 ) ) ;
#19264=CARTESIAN_POINT ( 'NONE',  ( -113.0906860500255391, -282.7326402546606232, -267.1428584951389098 ) ) ;
#19265=CARTESIAN_POINT ( 'NONE',  ( -64.38535207857050580, -292.0421006777201001, -198.2328756303478485 ) ) ;
#19266=CARTESIAN_POINT ( 'NONE',  ( 33.72264406068770626, -288.1068872051334324, -287.1523797545385719 ) ) ;
#19269=CARTESIAN_POINT ( 'NONE',  ( -76.58874877760752042, -208.1735614672835197, -353.4623537001039040 ) ) ;
#19270=CARTESIAN_POINT ( 'NONE',  ( -95.72720533505923868, -285.4044566034078798, -319.5121797396082570 ) ) ;
#19271=CARTESIAN_POINT ( 'NONE',  ( -85.33152481854864391, -281.1952119285918457, -330.4860931364850671 ) ) ;
#19273=CARTESIAN_POINT ( 'NONE',  ( 25.81839340915425396, -280.9827083662730161, -307.6773701161826011 ) ) ;
#19274=CARTESIAN_POINT ( 'NONE',  ( 34.16303839569806655, -275.5822831477111095, -299.0147507613526159 ) ) ;
#19275=CARTESIAN_POINT ( 'NONE',  ( -68.08211249619313321, -281.6477724909933045, -202.1192003733392824 ) ) ;
#19276=CARTESIAN_POINT ( 'NONE',  ( 155.4638711370593569, 204.8809718456330415, -215.8888951672738585 ) ) ;
#19277=CARTESIAN_POINT ( 'NONE',  ( -9.062181949930447900, -278.9895656462564943, -199.3760833295065424 ) ) ;
#19278=CARTESIAN_POINT ( 'NONE',  ( -97.06717561235315372, -283.1869425323889686, -225.5870810443808523 ) ) ;
#19279=CARTESIAN_POINT ( 'NONE',  ( -57.14748864760450431, -299.5603315045846102, -196.9464592911140528 ) ) ;
#19280=CARTESIAN_POINT ( 'NONE',  ( 6.104563476882358231, -294.9371745107561651, -329.1643668735893584 ) ) ;
#19282=CARTESIAN_POINT ( 'NONE',  ( -110.7370991443813892, -289.2982078910837345, -265.6876807222027992 ) ) ;
#19283=CARTESIAN_POINT ( 'NONE',  ( -56.89009676848863961, -277.9491165894031042, -344.7879520330303080 ) ) ;
#19284=CARTESIAN_POINT ( 'NONE',  ( -32.69103204684299868, -274.1123625625297109, -197.4968841856502593 ) ) ;
#19285=CARTESIAN_POINT ( 'NONE',  ( -41.16355307362950100, -272.9255770132322141, -193.7134674802490792 ) ) ;
#19287=CARTESIAN_POINT ( 'NONE',  ( 23.86119083419642095, -272.9626433515699659, -226.9893269079989295 ) ) ;
#19289=CARTESIAN_POINT ( 'NONE',  ( 35.99627554596227696, -282.6082011210353357, -268.5623309648966597 ) ) ;
#19290=CARTESIAN_POINT ( 'NONE',  ( 36.98867910418877614, -283.1115329481219192, -254.5202117064272329 ) ) ;
#19291=CARTESIAN_POINT ( 'NONE',  ( -88.97215051655771845, -283.1497116781166028, -322.1834016919127066 ) ) ;
#19292=CARTESIAN_POINT ( 'NONE',  ( 1.045801265805477387, -272.9737015388060968, -207.3306479573419665 ) ) ;
#19293=CARTESIAN_POINT ( 'NONE',  ( 7.876262782212916314, -282.5373320520805578, -211.4216398369878505 ) ) ;
#19294=CARTESIAN_POINT ( 'NONE',  ( 1.217866415617300913, -275.0073707914935426, -333.2212889912209448 ) ) ;
#19296=CARTESIAN_POINT ( 'NONE',  ( 33.15347234365612650, -276.3648219298077606, -250.0637712767699270 ) ) ;
#19298=CARTESIAN_POINT ( 'NONE',  ( -99.30372800989310633, -279.9599678542490437, -224.8981122928330194 ) ) ;
#19301=CARTESIAN_POINT ( 'NONE',  ( -57.45126543052634105, -287.6558475347466128, -197.2593302120670273 ) ) ;
#19302=CARTESIAN_POINT ( 'NONE',  ( -94.07423630157281025, -295.0966795284489876, -316.5762764205593953 ) ) ;
#19303=CARTESIAN_POINT ( 'NONE',  ( -69.32248810350432677, -288.8105656559068848, -340.3079334664897146 ) ) ;
#19304=CARTESIAN_POINT ( 'NONE',  ( 9.691465384147978313, -284.9497063866011786, -213.2134552761442592 ) ) ;
#19305=CARTESIAN_POINT ( 'NONE',  ( 34.57568247128498484, -285.9227753921196609, -254.7641631827181072 ) ) ;
#19306=CARTESIAN_POINT ( 'NONE',  ( -100.5657489523968593, -289.3147396615349862, -231.8813354662964912 ) ) ;
#19307=CARTESIAN_POINT ( 'NONE',  ( -95.42128366494856095, -285.1285621727255943, -315.2580422649932075 ) ) ;
#19308=CARTESIAN_POINT ( 'NONE',  ( -2.422104263145531622, -274.5899576302240916, -336.7359812670925976 ) ) ;
#19309=CARTESIAN_POINT ( 'NONE',  ( 11.57973657644783749, -285.1173745097558481, -211.8702211287368300 ) ) ;
#19310=CARTESIAN_POINT ( 'NONE',  ( -86.17973997582254242, -299.3754136886805668, -213.3729853843608737 ) ) ;
#19311=CARTESIAN_POINT ( 'NONE',  ( 36.30676224294442278, -285.7445636035419056, -285.3921665295383150 ) ) ;
#19312=CARTESIAN_POINT ( 'NONE',  ( 5.049630586105095631, -281.5824673427633229, -210.6419122963373525 ) ) ;
#19313=CARTESIAN_POINT ( 'NONE',  ( 15.41773474911120623, -290.3092396126820631, -323.9729513598685458 ) ) ;
#19316=CARTESIAN_POINT ( 'NONE',  ( -93.56345401848219012, -297.7740741019533743, -320.8623505491577816 ) ) ;
#19317=CARTESIAN_POINT ( 'NONE',  ( -57.63042878020125670, -277.7900246726454725, -198.1574606256745881 ) ) ;
#19318=CARTESIAN_POINT ( 'NONE',  ( -37.78382080134698384, -291.2439184691713763, -193.5238656197525700 ) ) ;
#19319=CARTESIAN_POINT ( 'NONE',  ( -109.8276189887545655, -295.1338145041859775, -256.4291338908207649 ) ) ;
#19320=CARTESIAN_POINT ( 'NONE',  ( 28.22890427824656356, -279.7879969233286488, -237.0557682084490807 ) ) ;
#19321=CARTESIAN_POINT ( 'NONE',  ( -49.07883902702410239, -271.9814315128986095, -196.8000682633288818 ) ) ;
#19322=CARTESIAN_POINT ( 'NONE',  ( 15.21654807871645509, -294.1283480494853393, -218.9182737601863664 ) ) ;
#19323=CARTESIAN_POINT ( 'NONE',  ( -106.6662871844225293, -299.4805209788416391, -237.0123917617630696 ) ) ;
#19324=CARTESIAN_POINT ( 'NONE',  ( -112.4531982868974751, -295.2018061084520468, -256.9085866942377834 ) ) ;
#19325=CARTESIAN_POINT ( 'NONE',  ( -6.233322651633932843, -292.8888790201270353, -339.6881896576142594 ) ) ;
#19326=CARTESIAN_POINT ( 'NONE',  ( -86.33473845658161849, -292.7818904339169990, -215.3829797432403552 ) ) ;
#19328=CARTESIAN_POINT ( 'NONE',  ( -89.93949945674523860, -292.0881928938936767, -219.5076694002517570 ) ) ;
#19330=CARTESIAN_POINT ( 'NONE',  ( -112.1741428937693712, -291.5513785533925670, -286.7353120116117680 ) ) ;
#19331=CARTESIAN_POINT ( 'NONE',  ( 10.42998291966162761, -280.4169801292837860, -328.7061751592140695 ) ) ;
#19332=CARTESIAN_POINT ( 'NONE',  ( 10.93080629530809667, -292.7419188015177838, -215.5326838798079621 ) ) ;
#19333=CARTESIAN_POINT ( 'NONE',  ( 22.87531297833881894, -280.9094443014819831, -222.3514976036543942 ) ) ;
#19334=CARTESIAN_POINT ( 'NONE',  ( -110.2060370730548726, -283.9059354087220299, -295.1911943630058204 ) ) ;
#19335=CARTESIAN_POINT ( 'NONE',  ( -98.06071458232067073, -287.9553087247246026, -314.1015993713901935 ) ) ;
#19336=CARTESIAN_POINT ( 'NONE',  ( -106.3711201022286588, -282.3308680365232135, -297.8105844061078074 ) ) ;
#19337=CARTESIAN_POINT ( 'NONE',  ( -2.687559918590475050, -278.9817740087083280, -202.3627121064109815 ) ) ;
#19338=CARTESIAN_POINT ( 'NONE',  ( -3.612852668795328182, -285.4071906515711134, -201.4709808852229855 ) ) ;
#19340=CARTESIAN_POINT ( 'NONE',  ( 4.945544221397195628, -294.2339694101602845, -209.8151869044908153 ) ) ;
#19341=CARTESIAN_POINT ( 'NONE',  ( 14.49686612503592720, -277.7654615448470281, -326.5702062463382163 ) ) ;
#19342=CARTESIAN_POINT ( 'NONE',  ( -43.21301939045737583, -276.7950518690103081, -343.1458354506034993 ) ) ;
#19343=CARTESIAN_POINT ( 'NONE',  ( -111.2327617711435721, -290.9904969963481562, -248.7021472365947545 ) ) ;
#19344=CARTESIAN_POINT ( 'NONE',  ( 16.77749209836053979, -280.3694807798769943, -323.1656105699629506 ) ) ;
#19345=CARTESIAN_POINT ( 'NONE',  ( 6.827659768009302965, -291.7289121733602428, -211.9447153736229836 ) ) ;
#19346=CARTESIAN_POINT ( 'NONE',  ( -111.2378981130450910, -294.3836093657660058, -283.4751613437791775 ) ) ;
#19349=CARTESIAN_POINT ( 'NONE',  ( 33.50419931762212400, -293.2952676138845050, -288.2174046506316358 ) ) ;
#19350=CARTESIAN_POINT ( 'NONE',  ( 120.8395553409046528, -296.8152984961567427, -195.3611179825600175 ) ) ;
#19351=CARTESIAN_POINT ( 'NONE',  ( -105.5795714935544112, -282.2666405000203440, -254.7536222014695397 ) ) ;
#19352=CARTESIAN_POINT ( 'NONE',  ( -90.55762577094819221, -294.8423941055107207, -325.7595832190785359 ) ) ;
#19353=CARTESIAN_POINT ( 'NONE',  ( 38.47453809775845457, -279.6866472146214164, -269.9608258604031334 ) ) ;
#19354=CARTESIAN_POINT ( 'NONE',  ( -1.217290840402611707, -287.8364056609063937, -202.9198448089321403 ) ) ;
#19355=CARTESIAN_POINT ( 'NONE',  ( 34.96007745442040715, -287.5195431365880836, -280.5244969956690397 ) ) ;
#19356=CARTESIAN_POINT ( 'NONE',  ( -62.00378850043031065, -278.8986713685884524, -339.8595075047044247 ) ) ;
#19357=CARTESIAN_POINT ( 'NONE',  ( -72.93049307174983653, -293.5461813092999819, -335.9903784861277245 ) ) ;
#19358=CARTESIAN_POINT ( 'NONE',  ( -111.2524442055989340, -298.2616144368424216, -274.2567464536628563 ) ) ;
#19359=CARTESIAN_POINT ( 'NONE',  ( -108.9910380518414712, -277.5566596118563325, -254.3818652144164787 ) ) ;
#19360=EDGE_LOOP ( 'NONE', ( #22867, #53348, #37110, #25874 ) ) ;
#19362=CARTESIAN_POINT ( 'NONE',  ( -92.68475354843974401, -295.4856827975393117, -323.8671057746762472 ) ) ;
#19363=CARTESIAN_POINT ( 'NONE',  ( -42.74448929455780899, -291.0408666532099460, -344.6564001954229752 ) ) ;
#19364=CARTESIAN_POINT ( 'NONE',  ( 36.32840533430368879, -295.3986030066924400, -289.8330459380111392 ) ) ;
#19367=CARTESIAN_POINT ( 'NONE',  ( 17.64932773812103406, -281.3482250297483347, -323.9983051005348784 ) ) ;
#19368=CARTESIAN_POINT ( 'NONE',  ( -107.0704490825032593, -296.7880487345041161, -302.7835539724968612 ) ) ;
#19369=CARTESIAN_POINT ( 'NONE',  ( -113.1325893188627560, -288.7171284882096529, -268.3632572824193403 ) ) ;
#19370=CARTESIAN_POINT ( 'NONE',  ( -87.45171586596606517, -297.7088026291820029, -211.8551487525683115 ) ) ;
#19374=CARTESIAN_POINT ( 'NONE',  ( -34.67152081584604417, -290.5392847426256822, -346.6210543625663831 ) ) ;
#19375=CARTESIAN_POINT ( 'NONE',  ( -99.90806341382572953, -275.6948066931273047, -220.5068182859052968 ) ) ;
#19378=CARTESIAN_POINT ( 'NONE',  ( -2.428998617669638538, -279.8503422498260989, -201.8306003024534050 ) ) ;
#19379=CARTESIAN_POINT ( 'NONE',  ( -112.2247868479535242, -286.5447593951460021, -270.9484879699466546 ) ) ;
#19381=CARTESIAN_POINT ( 'NONE',  ( -26.68518726441089228, -284.7597618869936014, -194.6440001154971924 ) ) ;
#19382=CARTESIAN_POINT ( 'NONE',  ( 25.34277220506094608, -272.9995144579653470, -229.4870998971572646 ) ) ;
#19383=CARTESIAN_POINT ( 'NONE',  ( -81.95316389797478962, -275.3594204872909472, -210.7050505781511447 ) ) ;
#19384=CARTESIAN_POINT ( 'NONE',  ( -85.63751318266520229, -287.8058732304746741, -327.0756974491847018 ) ) ;
#19385=CARTESIAN_POINT ( 'NONE',  ( -110.6265399009983241, -280.1673916383721803, -289.6379983987773699 ) ) ;
#19386=ORIENTED_EDGE ( 'NONE', *, *, #80976, .F. ) ;
#19387=CARTESIAN_POINT ( 'NONE',  ( -59.73363206496299682, -279.7539979123742455, -200.8268705012600606 ) ) ;
#19388=CARTESIAN_POINT ( 'NONE',  ( -14.26884904698354184, -279.7078560988997538, -200.9423640825450548 ) ) ;
#19389=CARTESIAN_POINT ( 'NONE',  ( 38.83223831995906039, -276.7490441371188581, -279.6965678161697610 ) ) ;
#19390=CARTESIAN_POINT ( 'NONE',  ( 38.40446978103273779, -280.1991257847736847, -258.5918179892675539 ) ) ;
#19391=CARTESIAN_POINT ( 'NONE',  ( 166.0191155783938370, 231.4420791936586852, -190.6152028106120895 ) ) ;
#19392=CARTESIAN_POINT ( 'NONE',  ( 37.05422437480636688, -276.2558900577091663, -251.4384693542097011 ) ) ;
#19393=CARTESIAN_POINT ( 'NONE',  ( 30.12263164617074551, -300.3064692177213715, -193.9343428704701182 ) ) ;
#19394=CARTESIAN_POINT ( 'NONE',  ( 35.77081079830085031, -283.8376638359844719, -253.6410175316879361 ) ) ;
#19397=CARTESIAN_POINT ( 'NONE',  ( 82.64890176555634582, -299.5541904835127980, -195.3611179825600175 ) ) ;
#19398=CARTESIAN_POINT ( 'NONE',  ( 34.29515255759648795, -288.4273135979447034, -254.7923218847039664 ) ) ;
#19399=CARTESIAN_POINT ( 'NONE',  ( 34.99012493043350958, -289.6089768121959764, -293.6437530815389323 ) ) ;
#19400=CARTESIAN_POINT ( 'NONE',  ( -96.64616049843958479, -289.3038380930856874, -313.1030604813448122 ) ) ;
#19401=CARTESIAN_POINT ( 'NONE',  ( -26.62347082025265976, -285.6925367351441878, -194.1194309527787993 ) ) ;
#19402=CARTESIAN_POINT ( 'NONE',  ( -46.98879273849259164, -155.5777431771304009, -365.1571803742538691 ) ) ;
#19403=CARTESIAN_POINT ( 'NONE',  ( -6.942361788622357643, -281.0463124202631775, -337.6231815527979734 ) ) ;
#19404=CARTESIAN_POINT ( 'NONE',  ( -74.18897684265721182, -287.4173580660720404, -205.9014855633704428 ) ) ;
#19405=CARTESIAN_POINT ( 'NONE',  ( -38.91914892066086651, -281.5521366313458884, -344.0501781010830200 ) ) ;
#19406=CARTESIAN_POINT ( 'NONE',  ( -96.01551138448773770, -280.4850423649531308, -226.0838409119601238 ) ) ;
#19407=CARTESIAN_POINT ( 'NONE',  ( -21.63368471006718252, -277.3377947579107854, -341.7661278118835071 ) ) ;
#19408=CARTESIAN_POINT ( 'NONE',  ( -93.31321642233871216, -288.6295358201517161, -322.7367040332125612 ) ) ;
#19409=CARTESIAN_POINT ( 'NONE',  ( -83.18774489038943898, -286.2452576912470477, -208.6319767399097316 ) ) ;
#19410=CARTESIAN_POINT ( 'NONE',  ( -93.38241247716482007, -284.3242155319110793, -323.0963244491782689 ) ) ;
#19411=CARTESIAN_POINT ( 'NONE',  ( 17.60625775002468529, -282.4045448989123201, -318.4206844552840039 ) ) ;
#19414=CARTESIAN_POINT ( 'NONE',  ( -102.1714003406963940, -292.9337910870783617, -231.0500252879517973 ) ) ;
#19415=CARTESIAN_POINT ( 'NONE',  ( -71.93421273947951988, -290.2893545709914065, -202.1069157976611734 ) ) ;
#19416=CARTESIAN_POINT ( 'NONE',  ( 20.04734331374150003, -273.9705821302050595, -224.8448262857601492 ) ) ;
#19417=CARTESIAN_POINT ( 'NONE',  ( -69.49287061192910642, -294.8128637054778665, -340.2297741149855028 ) ) ;
#19418=CARTESIAN_POINT ( 'NONE',  ( -108.0551838024495623, -289.3044209870867007, -249.5724138148768532 ) ) ;
#19420=CARTESIAN_POINT ( 'NONE',  ( -91.15926689724861376, -294.0695377649434477, -321.2448282055677851 ) ) ;
#19421=CARTESIAN_POINT ( 'NONE',  ( -82.78013088581576540, -290.8946686732883222, -328.0020714261202670 ) ) ;
#19423=CARTESIAN_POINT ( 'NONE',  ( -112.3687964989947545, -292.5770836642851691, -268.4322422422585532 ) ) ;
#19424=CARTESIAN_POINT ( 'NONE',  ( 18.08151948523178376, -290.8443932915548089, -219.5842024102376229 ) ) ;
#19425=CARTESIAN_POINT ( 'NONE',  ( -50.54293921849853177, -297.2207659589902846, -344.2423438634703530 ) ) ;
#19426=CARTESIAN_POINT ( 'NONE',  ( -77.18710288309884504, -286.4451848430729797, -208.8537922480863358 ) ) ;
#19427=CARTESIAN_POINT ( 'NONE',  ( -4.018081362540677048, -296.6139714307894906, -337.7516691833790219 ) ) ;
#19428=CARTESIAN_POINT ( 'NONE',  ( 37.09875191467167355, -277.3813898625871843, -258.5723126336488349 ) ) ;
#19429=CARTESIAN_POINT ( 'NONE',  ( 19.25122274158002966, -297.9409541251399673, -193.5300614419665806 ) ) ;
#19430=CARTESIAN_POINT ( 'NONE',  ( -26.90041023837674317, -275.1574151874874019, -343.6342609293431565 ) ) ;
#19431=CARTESIAN_POINT ( 'NONE',  ( -34.22911269578052185, -278.1714037116320242, -195.9734255393522631 ) ) ;
#19432=CARTESIAN_POINT ( 'NONE',  ( -105.7920830218455137, -274.1109254191138120, -243.7316835570631213 ) ) ;
#19433=CARTESIAN_POINT ( 'NONE',  ( -96.87449052283102446, -297.3766075508637527, -313.6402403777127574 ) ) ;
#19435=CARTESIAN_POINT ( 'NONE',  ( -109.4367199486425193, -297.5188125419746257, -257.9148396508234669 ) ) ;
#19437=CARTESIAN_POINT ( 'NONE',  ( -36.13893527901843328, -287.0572881008694139, -345.7195534182802703 ) ) ;
#19438=CARTESIAN_POINT ( 'NONE',  ( -68.28064516795458871, -273.4674572970430972, -204.2279701918880335 ) ) ;
#19439=CARTESIAN_POINT ( 'NONE',  ( -29.46293762432317820, -286.1493411985822490, -193.7652623413481194 ) ) ;
#19440=CARTESIAN_POINT ( 'NONE',  ( -51.68552784716350601, -288.8975643572458125, -345.9917923006224214 ) ) ;
#19441=CARTESIAN_POINT ( 'NONE',  ( -112.6667822721557286, -298.5770718032194964, -266.8378753867763749 ) ) ;
#19442=CARTESIAN_POINT ( 'NONE',  ( -64.25145865080580165, -293.4037719596401530, -340.2436272045648593 ) ) ;
#19443=CARTESIAN_POINT ( 'NONE',  ( 35.45280807396443379, -281.0616858521780728, -295.1255584212946133 ) ) ;
#19444=CARTESIAN_POINT ( 'NONE',  ( -37.30987171927208834, -289.5523547857347353, -195.3611179825600175 ) ) ;
#19445=CARTESIAN_POINT ( 'NONE',  ( 6.539178240135462339, -278.6479185318422651, -209.4745301464643319 ) ) ;
#19447=CARTESIAN_POINT ( 'NONE',  ( 14.35221991852950119, -287.1001778936119422, -322.4655240789244885 ) ) ;
#19449=CARTESIAN_POINT ( 'NONE',  ( -37.29156836245572038, -287.0513678757959610, -345.3611055862955936 ) ) ;
#19450=CARTESIAN_POINT ( 'NONE',  ( -55.51011055269275118, -299.4147173743010626, -198.7795694348580184 ) ) ;
#19451=CARTESIAN_POINT ( 'NONE',  ( 38.69370955966201819, -283.0792144695341790, -278.4380654923639895 ) ) ;
#19452=CARTESIAN_POINT ( 'NONE',  ( -59.63686598167379316, -295.7850441338677001, -198.3253160845473531 ) ) ;
#19453=CARTESIAN_POINT ( 'NONE',  ( 34.06519705922689667, -281.3513100447460147, -255.1339928361404645 ) ) ;
#19454=CARTESIAN_POINT ( 'NONE',  ( -83.57474877046688277, -274.8286870505082220, -213.1083440004505860 ) ) ;
#19455=CARTESIAN_POINT ( 'NONE',  ( 38.20092394607508623, -285.6113430087452798, -268.7405800503912019 ) ) ;
#19456=CARTESIAN_POINT ( 'NONE',  ( 35.72316715421460032, -283.3343134517385238, -253.3777033569439254 ) ) ;
#19458=CARTESIAN_POINT ( 'NONE',  ( -91.34096052969518098, -272.1812701167718842, -220.7612330509709011 ) ) ;
#19460=CARTESIAN_POINT ( 'NONE',  ( 204.4813248545303281, 292.6428223457351692, -53.99999999999219114 ) ) ;
#19461=CARTESIAN_POINT ( 'NONE',  ( -110.0211405059826575, -286.3118640372304640, -287.4329256685942369 ) ) ;
#19462=CARTESIAN_POINT ( 'NONE',  ( 36.60358173371529489, -272.6237833571633473, -234.7871824221999191 ) ) ;
#19463=CARTESIAN_POINT ( 'NONE',  ( -62.36309235902298553, -276.5665669388928904, -343.0677669624786859 ) ) ;
#19464=CARTESIAN_POINT ( 'NONE',  ( -112.1357604998202078, -289.1370197828583173, -255.7230979849308028 ) ) ;
#19465=CARTESIAN_POINT ( 'NONE',  ( -102.3740545431648030, -285.6030531752517732, -305.1323425053922165 ) ) ;
#19466=CARTESIAN_POINT ( 'NONE',  ( 36.44231860042102511, -277.1322467691106795, -268.8252165147472397 ) ) ;
#19467=CARTESIAN_POINT ( 'NONE',  ( -66.33572811649945322, -284.8496516571270831, -341.0713932220160132 ) ) ;
#19468=CARTESIAN_POINT ( 'NONE',  ( -7.103839026762195807, -281.4413011762461565, -337.2539166903729893 ) ) ;
#19469=CARTESIAN_POINT ( 'NONE',  ( -73.10523034926555397, -281.5781949023370885, -204.4371423984183878 ) ) ;
#19470=CARTESIAN_POINT ( 'NONE',  ( 2.416184001802894610, -274.7362494710105238, -204.4193963336869047 ) ) ;
#19471=CARTESIAN_POINT ( 'NONE',  ( -7.886600221975030856, -276.5100736484404251, -341.5188989344426318 ) ) ;
#19472=CARTESIAN_POINT ( 'NONE',  ( -93.25646696972620475, -297.7843342022456454, -319.5022723105683440 ) ) ;
#19475=CARTESIAN_POINT ( 'NONE',  ( -111.9910846304421881, -294.5233313311862275, -283.6109018952587348 ) ) ;
#19476=CARTESIAN_POINT ( 'NONE',  ( 25.42523679733339748, -275.5734822009889626, -307.7549686876437818 ) ) ;
#19477=CARTESIAN_POINT ( 'NONE',  ( -20.60763997381464918, -299.3367160135730387, -193.6672397974564035 ) ) ;
#19478=CARTESIAN_POINT ( 'NONE',  ( -22.27515888739961980, -288.0077523746222710, -197.8449204549039280 ) ) ;
#19479=CARTESIAN_POINT ( 'NONE',  ( 35.61833481942879587, -294.7890707294258164, -248.0107029232511593 ) ) ;
#19480=CARTESIAN_POINT ( 'NONE',  ( 37.03272232231700656, -294.5265677265944646, -252.0184353741070140 ) ) ;
#19482=CARTESIAN_POINT ( 'NONE',  ( -94.86504419410113087, -293.2149144735826098, -222.4757380611491158 ) ) ;
#19483=CARTESIAN_POINT ( 'NONE',  ( -2.267823063134530859, -278.5172269377239331, -204.2417290563731740 ) ) ;
#19484=CARTESIAN_POINT ( 'NONE',  ( -52.13702688884777814, -281.7815889881048292, -197.3534978758159468 ) ) ;
#19485=CARTESIAN_POINT ( 'NONE',  ( -72.83224060477833461, -293.6059097861643181, -335.8106439962826926 ) ) ;
#19486=CARTESIAN_POINT ( 'NONE',  ( 0.2759929415788082152, -284.4171896256192440, -336.1424722854899869 ) ) ;
#19487=CARTESIAN_POINT ( 'NONE',  ( -108.3245363648242972, -283.7133148990215545, -252.0400090034268885 ) ) ;
#19488=CARTESIAN_POINT ( 'NONE',  ( -93.21478779330486475, -240.8791580765806088, -341.0619996075755012 ) ) ;
#19490=CARTESIAN_POINT ( 'NONE',  ( -74.72729022312158520, -285.2062956943942709, -207.6362812747704538 ) ) ;
#19492=CARTESIAN_POINT ( 'NONE',  ( -4.284572199490292554, -283.7062449515055960, -339.5761198286045897 ) ) ;
#19493=CARTESIAN_POINT ( 'NONE',  ( -27.29146742889274435, -274.5165431070660702, -197.9839973314861368 ) ) ;
#19494=CARTESIAN_POINT ( 'NONE',  ( 31.07408505274378996, -285.9014066330980199, -235.9040569418474718 ) ) ;
#19495=CARTESIAN_POINT ( 'NONE',  ( 26.07943445700025364, -281.9201485474387141, -227.0181869501322467 ) ) ;
#19496=CARTESIAN_POINT ( 'NONE',  ( -74.97723650541998097, -279.0641608532977784, -336.7408901622046073 ) ) ;
#19497=CARTESIAN_POINT ( 'NONE',  ( -36.76166467069850086, -280.7106732390200818, -193.4522099878877555 ) ) ;
#19498=CARTESIAN_POINT ( 'NONE',  ( -67.68488546085839630, -277.1237833571632905, -207.2794874003663779 ) ) ;
#19499=CARTESIAN_POINT ( 'NONE',  ( 175.0256770085078983, 242.8924757603117541, -179.7605988551675580 ) ) ;
#19501=CARTESIAN_POINT ( 'NONE',  ( -5.778309749577410059, -276.4682931798193408, -202.5099513130991511 ) ) ;
#19502=CARTESIAN_POINT ( 'NONE',  ( 179.5181012596348751, 254.3142353492114296, -166.5901205928782645 ) ) ;
#19503=CARTESIAN_POINT ( 'NONE',  ( -30.07778042622149073, -278.1644878974050812, -196.0191018990759630 ) ) ;
#19504=CARTESIAN_POINT ( 'NONE',  ( 22.29859497045398342, -294.6738642988329957, -223.2552068712512323 ) ) ;
#19505=CARTESIAN_POINT ( 'NONE',  ( -53.17953288726015870, -294.6090767794040062, -341.7788244049817195 ) ) ;
#19506=CARTESIAN_POINT ( 'NONE',  ( -66.98593661265492472, -291.1815266414670873, -199.3629057052757503 ) ) ;
#19508=CARTESIAN_POINT ( 'NONE',  ( -101.0483277147252466, -295.6864341085647538, -228.1464024302122198 ) ) ;
#19509=CARTESIAN_POINT ( 'NONE',  ( 20.12372798844755906, -286.5996363189235012, -316.6662471702024391 ) ) ;
#19510=CARTESIAN_POINT ( 'NONE',  ( 36.87787846106154888, -295.4535302682090787, -273.5182665011015501 ) ) ;
#19511=CARTESIAN_POINT ( 'NONE',  ( -106.0317635033066210, -286.2138949110586736, -244.2284053279668967 ) ) ;
#19513=CARTESIAN_POINT ( 'NONE',  ( -109.2576333635352483, -291.8357203872217269, -243.3596399460035684 ) ) ;
#19514=CARTESIAN_POINT ( 'NONE',  ( 18.54547584344189204, -282.7126212731938040, -317.4402051643497771 ) ) ;
#19515=CARTESIAN_POINT ( 'NONE',  ( -112.2202928446892116, -295.1439084619268556, -286.5229580100850626 ) ) ;
#19516=CARTESIAN_POINT ( 'NONE',  ( -97.15791443741044020, -290.7068416908382460, -318.6123459103395703 ) ) ;
#19517=CARTESIAN_POINT ( 'NONE',  ( -100.6264103876781206, -290.4661746272823848, -314.1169444588870761 ) ) ;
#19518=CARTESIAN_POINT ( 'NONE',  ( 35.27417659623907298, -287.6201736092147598, -262.8821840977455508 ) ) ;
#19521=CARTESIAN_POINT ( 'NONE',  ( -65.12808339599854435, -297.2717749781036787, -340.8607280826007013 ) ) ;
#19522=CARTESIAN_POINT ( 'NONE',  ( -111.7905790197203828, -295.4588520593165413, -252.7354915619162057 ) ) ;
#19523=CARTESIAN_POINT ( 'NONE',  ( 19.86730956892184352, -279.9670414364985618, -224.6387202057887009 ) ) ;
#19525=CARTESIAN_POINT ( 'NONE',  ( 38.12078599941734325, -275.2475281872420965, -285.3591208794525755 ) ) ;
#19527=CARTESIAN_POINT ( 'NONE',  ( -110.7390068134509562, -295.1254274995856122, -263.2133351378632824 ) ) ;
#19528=CARTESIAN_POINT ( 'NONE',  ( -37.79390056430135303, -278.9182544319880890, -344.6076084687080652 ) ) ;
#19529=CARTESIAN_POINT ( 'NONE',  ( 36.61092313206808058, -273.6004808806676465, -263.3268763405372965 ) ) ;
#19530=CARTESIAN_POINT ( 'NONE',  ( -66.19517610796971496, -296.6435585387627043, -337.8489496966423076 ) ) ;
#19531=CARTESIAN_POINT ( 'NONE',  ( -106.1005258454177778, -297.9711562326219791, -244.7892399344289345 ) ) ;
#19533=CARTESIAN_POINT ( 'NONE',  ( -92.10772536110540898, -297.4187805553817157, -323.3434064864345601 ) ) ;
#19534=CARTESIAN_POINT ( 'NONE',  ( -94.75772925859425300, -271.2447616858585207, -221.5375050123102767 ) ) ;
#19535=CARTESIAN_POINT ( 'NONE',  ( -2.397997746604971780, -293.1788268533762221, -206.1376338038719780 ) ) ;
#19536=CARTESIAN_POINT ( 'NONE',  ( -77.56214637827635272, -290.0753201204041716, -208.7357123471115870 ) ) ;
#19538=CARTESIAN_POINT ( 'NONE',  ( 29.89070456516675378, -275.5579666380244817, -232.8439520388284620 ) ) ;
#19539=CARTESIAN_POINT ( 'NONE',  ( -107.8571847730526230, -297.1364233326436874, -251.3483811165647239 ) ) ;
#19540=CARTESIAN_POINT ( 'NONE',  ( 19.80198164101667047, -282.8542852446947791, -221.2191436886357394 ) ) ;
#19541=CARTESIAN_POINT ( 'NONE',  ( 16.88547115480753291, -279.4893537735560471, -216.3172659066114534 ) ) ;
#19542=CARTESIAN_POINT ( 'NONE',  ( -96.98060673086467887, -277.2482760934615840, -318.9256753709169629 ) ) ;
#19543=CARTESIAN_POINT ( 'NONE',  ( 35.41795174450378880, -279.6646591839970597, -247.7232409878020576 ) ) ;
#19544=CARTESIAN_POINT ( 'NONE',  ( 25.69297347687545141, -281.2595026035443766, -307.5992111682854215 ) ) ;
#19545=CARTESIAN_POINT ( 'NONE',  ( 34.43286967942899679, -279.2646916444378462, -248.0353580658202475 ) ) ;
#19546=CARTESIAN_POINT ( 'NONE',  ( 13.92001354922727963, -273.3634149119303629, -217.5632806479824239 ) ) ;
#19547=CARTESIAN_POINT ( 'NONE',  ( -106.8067075046749466, -280.9225857543624443, -241.9483524703122441 ) ) ;
#19550=CARTESIAN_POINT ( 'NONE',  ( -80.03688364510111342, -295.7232943209882023, -207.4401271544244594 ) ) ;
#19551=CARTESIAN_POINT ( 'NONE',  ( -53.38931786843857452, -291.8519327235883338, -194.9974311095321582 ) ) ;
#19552=CARTESIAN_POINT ( 'NONE',  ( 26.11511654838982111, -278.0943193263464082, -310.7476310939799760 ) ) ;
#19553=CARTESIAN_POINT ( 'NONE',  ( -79.97149403564445436, -271.4756853547752939, -208.5914724473852289 ) ) ;
#19555=CARTESIAN_POINT ( 'NONE',  ( -94.23407710033788476, -285.7869239796958141, -320.0860779359610433 ) ) ;
#19557=CARTESIAN_POINT ( 'NONE',  ( 37.64557036340986684, -285.5121675678184374, -267.2598578389902286 ) ) ;
#19559=CARTESIAN_POINT ( 'NONE',  ( 33.49591756564610989, -292.6000761556006751, -289.6224664639239563 ) ) ;
#19560=CARTESIAN_POINT ( 'NONE',  ( 26.01708183997713419, -285.1676366962180964, -231.6761050384101566 ) ) ;
#19561=CARTESIAN_POINT ( 'NONE',  ( -75.31871349344845612, -193.4224457575235192, -358.3059354159982490 ) ) ;
#19562=CARTESIAN_POINT ( 'NONE',  ( -79.08344145442049467, -293.6145419377324401, -332.7345953412741437 ) ) ;
#19563=CARTESIAN_POINT ( 'NONE',  ( -82.84675689506562435, -283.9226769932094498, -209.0416881251521488 ) ) ;
#19564=CARTESIAN_POINT ( 'NONE',  ( -70.11369419273363235, -281.2131257202270262, -204.2227143297434395 ) ) ;
#19565=CARTESIAN_POINT ( 'NONE',  ( 1.308016098052928067, -287.7614439222979854, -204.2080636061183156 ) ) ;
#19566=CARTESIAN_POINT ( 'NONE',  ( 3.299190660261174024, -278.8297374877788570, -206.0938766645446663 ) ) ;
#19567=CARTESIAN_POINT ( 'NONE',  ( -106.0325700772870476, -290.2230626197979291, -295.0707190643522040 ) ) ;
#19568=CARTESIAN_POINT ( 'NONE',  ( -59.93163074521979183, -281.1790406629697827, -200.2711736610520461 ) ) ;
#19569=CARTESIAN_POINT ( 'NONE',  ( -16.88634231863705182, -281.1260295508619151, -200.1173989507307169 ) ) ;
#19570=CARTESIAN_POINT ( 'NONE',  ( -26.87505113223141251, -288.1643779550932436, -195.6839948042730555 ) ) ;
#19572=CARTESIAN_POINT ( 'NONE',  ( -26.99651961282917867, -274.1800832024772490, -194.0058057105406988 ) ) ;
#19573=CARTESIAN_POINT ( 'NONE',  ( -103.0800100968285875, -292.0591761065450669, -305.8305225488045380 ) ) ;
#19575=CARTESIAN_POINT ( 'NONE',  ( 44.71564893372296723, -296.0519495502701943, -270.3284710469131937 ) ) ;
#19576=ORIENTED_EDGE ( 'NONE', *, *, #5059, .T. ) ;
#19577=CARTESIAN_POINT ( 'NONE',  ( -38.30767883862273493, -272.0399123529101075, -195.2006542008588212 ) ) ;
#19579=CARTESIAN_POINT ( 'NONE',  ( 0.1291653543521297798, -292.9618621637017100, -336.7265308687156562 ) ) ;
#19580=CARTESIAN_POINT ( 'NONE',  ( -108.0365170528754959, -272.1483792230273480, -251.5623744590946274 ) ) ;
#19581=CARTESIAN_POINT ( 'NONE',  ( -61.46386170854030695, -290.8913998111416959, -339.9946520913386507 ) ) ;
#19582=CARTESIAN_POINT ( 'NONE',  ( -29.31275414760042608, -284.7093371208448502, -343.9888821885774632 ) ) ;
#19583=CARTESIAN_POINT ( 'NONE',  ( -41.70860172938049715, -290.5313889818283428, -346.6601254359052859 ) ) ;
#19584=CARTESIAN_POINT ( 'NONE',  ( -43.12818387945036136, -290.4389445989027649, -346.6488291725361250 ) ) ;
#19585=CARTESIAN_POINT ( 'NONE',  ( 8.119539619085845317, -288.6734769072125459, -210.6442281288526317 ) ) ;
#19586=CARTESIAN_POINT ( 'NONE',  ( -14.22978131563478854, -280.5103562792286311, -196.8556491659560095 ) ) ;
#19587=CARTESIAN_POINT ( 'NONE',  ( -105.8708425130099187, -294.2168953295993674, -302.1898917438289800 ) ) ;
#19588=CARTESIAN_POINT ( 'NONE',  ( -86.10400932912597227, -283.5404450889965915, -329.9533759181841788 ) ) ;
#19589=CARTESIAN_POINT ( 'NONE',  ( -4.787412233589957822, -276.3459418369423020, -203.6306191924289521 ) ) ;
#19591=CARTESIAN_POINT ( 'NONE',  ( 27.36219212280431989, -278.4805209788416391, -301.4846348637938149 ) ) ;
#19592=CARTESIAN_POINT ( 'NONE',  ( 38.54379683051755023, -273.7307461590430648, -265.5268812043017306 ) ) ;
#19594=CARTESIAN_POINT ( 'NONE',  ( 35.58166762261365079, -281.0006054385590915, -265.8699179869444720 ) ) ;
#19595=CARTESIAN_POINT ( 'NONE',  ( -51.22551418447954319, -278.4309355136653608, -345.6953626843069856 ) ) ;
#19596=AXIS2_PLACEMENT_3D ( 'NONE', #2561, #53195, #87774 ) ;
#19597=CARTESIAN_POINT ( 'NONE',  ( -105.2184239451338925, -284.0765554432099975, -234.3924822740572438 ) ) ;
#19598=CARTESIAN_POINT ( 'NONE',  ( -4.401955851565386268, -294.2524402574632632, -204.0676892681283618 ) ) ;
#19599=CARTESIAN_POINT ( 'NONE',  ( -38.36729687786588272, -275.6396185786705360, -194.1680174449055869 ) ) ;
#19600=CARTESIAN_POINT ( 'NONE',  ( -92.82613347742224619, -274.5919936852125716, -217.6658532834244681 ) ) ;
#19602=CARTESIAN_POINT ( 'NONE',  ( -11.25602427284302109, -276.5358373546932853, -338.5413021982215014 ) ) ;
#19603=CARTESIAN_POINT ( 'NONE',  ( -58.91296420194156980, -297.3320423923565841, -342.0180017439558924 ) ) ;
#19604=CARTESIAN_POINT ( 'NONE',  ( -70.77931714641178473, -283.6099794526190294, -203.3994268745634884 ) ) ;
#19605=CARTESIAN_POINT ( 'NONE',  ( 8.841633256664769291, -292.3325536065581218, -208.7085176790063485 ) ) ;
#19606=CARTESIAN_POINT ( 'NONE',  ( 30.59323416358538594, -273.1629794480649593, -239.3055581775890062 ) ) ;
#19607=CARTESIAN_POINT ( 'NONE',  ( 29.66898077533889477, -289.6277234983708695, -306.7483626064407076 ) ) ;
#19608=CARTESIAN_POINT ( 'NONE',  ( 35.95039856128092737, -292.5139160932710638, -273.5159278391927842 ) ) ;
#19610=CARTESIAN_POINT ( 'NONE',  ( -40.58907249422940566, -290.5868279356390076, -194.0062991542219493 ) ) ;
#19611=CARTESIAN_POINT ( 'NONE',  ( -94.12340507806628409, -289.5696727001651425, -316.2732674622867535 ) ) ;
#19613=CARTESIAN_POINT ( 'NONE',  ( 37.20719950797992226, -288.8584859785029266, -288.4153615057131219 ) ) ;
#19614=CARTESIAN_POINT ( 'NONE',  ( -99.19074347219216747, -278.3484204529441399, -309.2728663125286630 ) ) ;
#19616=CARTESIAN_POINT ( 'NONE',  ( 6.426266550188667104, -293.3934825830512523, -333.4008727872264899 ) ) ;
#19617=CARTESIAN_POINT ( 'NONE',  ( -65.84729576893857939, -286.3403113424697608, -198.9274896755308077 ) ) ;
#19618=CARTESIAN_POINT ( 'NONE',  ( -93.90708481666278828, -285.5971835479311949, -218.0709097067394282 ) ) ;
#19619=CARTESIAN_POINT ( 'NONE',  ( 34.72511216175007576, -282.0406160159020033, -282.1281079625403549 ) ) ;
#19620=CARTESIAN_POINT ( 'NONE',  ( 185.4827870066121420, 263.6036262534566958, -153.3731815501813287 ) ) ;
#19621=CARTESIAN_POINT ( 'NONE',  ( 43.70754100293377320, 12.83641530529500230, -330.7637548252565693 ) ) ;
#19622=CARTESIAN_POINT ( 'NONE',  ( 101.8919747252719503, 115.3001919161196298, -279.7615209532445419 ) ) ;
#19623=CARTESIAN_POINT ( 'NONE',  ( 26.78297338306001407, -274.2680019390987241, -235.0329552948199137 ) ) ;
#19624=CARTESIAN_POINT ( 'NONE',  ( 19.41220318830806590, -275.1269586707234112, -316.7837016143473079 ) ) ;
#19625=CARTESIAN_POINT ( 'NONE',  ( -97.29444852694773260, -296.7065741132399808, -222.1408435847179419 ) ) ;
#19626=CARTESIAN_POINT ( 'NONE',  ( -104.5998066112789644, -261.3044276662151333, -315.9010574050290643 ) ) ;
#19627=CARTESIAN_POINT ( 'NONE',  ( 30.10038376170000518, -274.7081494616471105, -306.5958297535347583 ) ) ;
#19628=CARTESIAN_POINT ( 'NONE',  ( -59.80422781972996660, -275.5174150529499002, -199.7850559432307591 ) ) ;
#19630=CARTESIAN_POINT ( 'NONE',  ( -99.73731463604903524, -298.0877647455494071, -225.6441468924830644 ) ) ;
#19631=CARTESIAN_POINT ( 'NONE',  ( 34.34575610701025994, -288.2312402561335034, -284.5289057701014599 ) ) ;
#19632=CARTESIAN_POINT ( 'NONE',  ( -94.52455482727145863, -296.6569330555036572, -321.7059550712958753 ) ) ;
#19633=CARTESIAN_POINT ( 'NONE',  ( -106.4607857110296152, -297.4788059414447048, -236.5664599545320641 ) ) ;
#19634=CARTESIAN_POINT ( 'NONE',  ( 34.32478059344524723, -293.9020571189629436, -284.2505220560532848 ) ) ;
#19636=CARTESIAN_POINT ( 'NONE',  ( 27.25848415957279869, -276.9497656794484897, -231.0676451195035099 ) ) ;
#19638=CARTESIAN_POINT ( 'NONE',  ( -19.76418420593281766, -279.7798115852958745, -195.4027331056911123 ) ) ;
#19639=CARTESIAN_POINT ( 'NONE',  ( -32.39272349485402458, -277.9296210395533535, -343.4791318620034986 ) ) ;
#19640=CARTESIAN_POINT ( 'NONE',  ( -32.76631449444165156, -275.8691727412134469, -194.4993442762985012 ) ) ;
#19641=CARTESIAN_POINT ( 'NONE',  ( -74.54654198849124214, -275.5647117204638334, -335.8913136616171187 ) ) ;
#19642=CARTESIAN_POINT ( 'NONE',  ( -92.82718225066639661, -297.8803225160447710, -222.7471772407489823 ) ) ;
#19643=CARTESIAN_POINT ( 'NONE',  ( -94.41092623939734096, -294.4743406805955033, -316.8403549952678873 ) ) ;
#19645=CARTESIAN_POINT ( 'NONE',  ( 12.94721008102246174, -281.2250624549287181, -212.1326677795434250 ) ) ;
#19646=CARTESIAN_POINT ( 'NONE',  ( 3.135869998262936331, -276.6581652179443722, -331.1111494324139812 ) ) ;
#19647=CARTESIAN_POINT ( 'NONE',  ( 38.86506681061069202, -286.1445945879853525, -263.0213388523831668 ) ) ;
#19648=CARTESIAN_POINT ( 'NONE',  ( -108.2203180557378772, -274.8696739446943411, -245.8412858368496927 ) ) ;
#19649=CARTESIAN_POINT ( 'NONE',  ( 82.68073018288104947, -297.0543924324409204, -195.4120394483015559 ) ) ;
#19650=CARTESIAN_POINT ( 'NONE',  ( 14.18988546296487741, -287.5023562168280478, -322.2947045452755219 ) ) ;
#19651=CARTESIAN_POINT ( 'NONE',  ( 22.15676834298203701, -279.1830263801064120, -226.3181223125586428 ) ) ;
#19652=CARTESIAN_POINT ( 'NONE',  ( -36.98741841384914864, -278.6314003859331478, -196.7727397997874448 ) ) ;
#19653=CARTESIAN_POINT ( 'NONE',  ( -89.92853646524764599, -281.8811752907210462, -323.1206733906225850 ) ) ;
#19654=CARTESIAN_POINT ( 'NONE',  ( -14.24238930478394849, -288.3517357250240138, -198.9533476307918249 ) ) ;
#19655=CARTESIAN_POINT ( 'NONE',  ( -108.1996132146635432, -279.5057944259626765, -289.4997349308646903 ) ) ;
#19657=CARTESIAN_POINT ( 'NONE',  ( -72.51880510702238780, -293.5867174665395964, -204.1078535119520438 ) ) ;
#19658=CARTESIAN_POINT ( 'NONE',  ( -92.61253242368304939, -276.0698836054360186, -322.5817248135517730 ) ) ;
#19660=CARTESIAN_POINT ( 'NONE',  ( -5.013548982505705354, -277.2663799546780297, -335.9401358482916748 ) ) ;
#19661=CARTESIAN_POINT ( 'NONE',  ( 18.44050481977730982, -284.2537714581124533, -320.8195784446700145 ) ) ;
#19663=CARTESIAN_POINT ( 'NONE',  ( -111.2369507814203757, -292.6740740063152657, -254.5263891447043818 ) ) ;
#19664=CARTESIAN_POINT ( 'NONE',  ( -103.6660590602784850, -295.0174025927381081, -235.2361043553986804 ) ) ;
#19665=CARTESIAN_POINT ( 'NONE',  ( -100.8572357993364363, -284.3218524460170897, -227.0243940207085700 ) ) ;
#19667=CARTESIAN_POINT ( 'NONE',  ( -81.35302854835673259, -272.1246130319072449, -211.4394216006893430 ) ) ;
#19668=CARTESIAN_POINT ( 'NONE',  ( -36.16315086508631538, -290.2066310600814063, -196.1225827854780732 ) ) ;
#19671=CARTESIAN_POINT ( 'NONE',  ( -66.73036770220565472, -290.1539178826674288, -199.9408512141963001 ) ) ;
#19672=CARTESIAN_POINT ( 'NONE',  ( 38.33619385700066573, -285.8787378740418035, -277.2043901635170755 ) ) ;
#19674=CARTESIAN_POINT ( 'NONE',  ( -110.9799068465407856, -285.9699637215548478, -270.9318380093532710 ) ) ;
#19675=CARTESIAN_POINT ( 'NONE',  ( -71.26214713705579129, -286.3950412505004124, -205.5382439172087743 ) ) ;
#19676=CARTESIAN_POINT ( 'NONE',  ( -22.54204002674223162, -294.2204577724324395, -196.4203591817009169 ) ) ;
#19677=CARTESIAN_POINT ( 'NONE',  ( -7.172545680384787126, -274.7393621255194489, -339.6509040317794756 ) ) ;
#19678=CARTESIAN_POINT ( 'NONE',  ( 36.56436033103000227, -275.6132200038420024, -248.6426118559175507 ) ) ;
#19679=CARTESIAN_POINT ( 'NONE',  ( -25.22775416250377134, -290.2852867372482137, -195.7785026567699447 ) ) ;
#19680=CARTESIAN_POINT ( 'NONE',  ( -107.4191222988419696, -278.9614488591267332, -238.3242045949060923 ) ) ;
#19681=CARTESIAN_POINT ( 'NONE',  ( -104.2311226638829709, -298.0914451866808577, -303.6086752717274067 ) ) ;
#19684=CARTESIAN_POINT ( 'NONE',  ( -94.49505170464325943, -283.8862425032945680, -224.1379548612009671 ) ) ;
#19685=CARTESIAN_POINT ( 'NONE',  ( -7.015099983241920079, -278.4498802124176109, -201.7520392936258702 ) ) ;
#19687=CARTESIAN_POINT ( 'NONE',  ( -21.47985050700745546, -272.7318698313854952, -195.7212527797362611 ) ) ;
#19688=CARTESIAN_POINT ( 'NONE',  ( -85.17820155550340644, -277.0817093105747517, -325.7053148123472965 ) ) ;
#19689=CARTESIAN_POINT ( 'NONE',  ( 8.676076768217118484, -295.9287765001250250, -327.9860053392569625 ) ) ;
#19690=CARTESIAN_POINT ( 'NONE',  ( 37.95382898646369085, -280.2896231767836639, -255.7982952493898949 ) ) ;
#19691=CARTESIAN_POINT ( 'NONE',  ( 18.15855984532634793, -295.1718741233734136, -318.1623481909813336 ) ) ;
#19692=CARTESIAN_POINT ( 'NONE',  ( -88.26462543217742507, -297.0626568651287016, -327.5299037707362118 ) ) ;
#19693=CARTESIAN_POINT ( 'NONE',  ( -35.14562830694016071, -297.9137171610188943, -197.3611822273222458 ) ) ;
#19694=CARTESIAN_POINT ( 'NONE',  ( -112.2446338966031192, -292.6130086750177952, -265.6342764491004118 ) ) ;
#19695=CARTESIAN_POINT ( 'NONE',  ( -4.775876822855616766, -286.6360087948301612, -200.5867161077590026 ) ) ;
#19696=CARTESIAN_POINT ( 'NONE',  ( 32.58286245647676083, -273.3131932041474670, -241.0559906015652700 ) ) ;
#19697=CARTESIAN_POINT ( 'NONE',  ( -36.08897095696743662, -288.8702068675487453, -347.3640372530098261 ) ) ;
#19698=CARTESIAN_POINT ( 'NONE',  ( -24.62031947533433396, -282.1951881461678795, -196.8083255521464423 ) ) ;
#19700=CARTESIAN_POINT ( 'NONE',  ( -30.49739542974624129, -285.1994256252635296, -197.3953836105832806 ) ) ;
#19701=CARTESIAN_POINT ( 'NONE',  ( -83.02736304058474559, -289.4271986102591541, -210.8160960141771909 ) ) ;
#19702=CARTESIAN_POINT ( 'NONE',  ( 198.7213489544213303, 274.9184959104715631, -125.0903475807052416 ) ) ;
#19703=CARTESIAN_POINT ( 'NONE',  ( -10.72171321864602156, -285.9165616421683467, -202.3081449986320024 ) ) ;
#19705=CARTESIAN_POINT ( 'NONE',  ( 37.63830155107445563, -282.7006045018844702, -286.8784615048901969 ) ) ;
#19706=CARTESIAN_POINT ( 'NONE',  ( -114.0168623531891967, -289.5644021979895228, -274.0678294754696935 ) ) ;
#19707=CARTESIAN_POINT ( 'NONE',  ( -42.39753414699718093, -281.5895124599226733, -194.3290263488046321 ) ) ;
#19708=CARTESIAN_POINT ( 'NONE',  ( -99.85575994222260476, -280.4546632004311846, -226.2556693533755094 ) ) ;
#19709=CARTESIAN_POINT ( 'NONE',  ( 34.06564199394210846, -281.1846570255385132, -255.1360791399640675 ) ) ;
#19710=CARTESIAN_POINT ( 'NONE',  ( 23.07765528434189051, -276.9462939751554131, -225.9257475807246465 ) ) ;
#19711=CARTESIAN_POINT ( 'NONE',  ( -41.94556103032653027, -295.1085237700092421, -347.2757548767604590 ) ) ;
#19712=CARTESIAN_POINT ( 'NONE',  ( -82.70917201603603530, -289.4491225278515003, -211.0197694380165387 ) ) ;
#19713=CARTESIAN_POINT ( 'NONE',  ( -71.79818029325973328, -296.5058242797296089, -205.6400064961015630 ) ) ;
#19716=CARTESIAN_POINT ( 'NONE',  ( -79.16589712348211094, -285.5414983966610976, -331.9407472564299155 ) ) ;
#19717=CARTESIAN_POINT ( 'NONE',  ( -110.1206748168517606, -296.1326706596463509, -276.8973139176134168 ) ) ;
#19718=CARTESIAN_POINT ( 'NONE',  ( 30.61860236383399680, -294.1701763916955201, -234.7096720974109871 ) ) ;
#19719=CARTESIAN_POINT ( 'NONE',  ( -78.42707957339293046, -284.2729618792450310, -330.8250267528971449 ) ) ;
#19720=ADVANCED_FACE ( 'NONE', ( #20703 ), #78009, .T. ) ;
#19721=CARTESIAN_POINT ( 'NONE',  ( 21.67766519286977811, -273.9486810173527260, -221.2741061470665329 ) ) ;
#19722=CARTESIAN_POINT ( 'NONE',  ( -72.13357699223674047, -292.2556236867211510, -201.7692956589353912 ) ) ;
#19723=CARTESIAN_POINT ( 'NONE',  ( -112.9178208589332115, -282.7684858132503791, -264.3227084533477296 ) ) ;
#19725=CARTESIAN_POINT ( 'NONE',  ( -39.21543250222599397, -292.3625520495683645, -193.3920377942747280 ) ) ;
#19726=CARTESIAN_POINT ( 'NONE',  ( 33.10343484458137198, -288.1415686587847063, -289.7730104989897200 ) ) ;
#19728=CARTESIAN_POINT ( 'NONE',  ( 144.2857639756989272, -299.5541904835127980, -195.3611179825600175 ) ) ;
#19729=CARTESIAN_POINT ( 'NONE',  ( 138.7881348363077052, 178.2172623047512161, -238.2660695523903485 ) ) ;
#19731=CARTESIAN_POINT ( 'NONE',  ( 21.09167699642706140, -283.7390007671057788, -319.4350233954951364 ) ) ;
#19732=CARTESIAN_POINT ( 'NONE',  ( 31.95455697924147032, -285.4809262143061801, -303.7686719486574702 ) ) ;
#19734=CARTESIAN_POINT ( 'NONE',  ( 23.94849149654265119, -279.9161214585595872, -230.0484276068459621 ) ) ;
#19735=CARTESIAN_POINT ( 'NONE',  ( -59.66293500783951487, -277.0003116746102592, -344.0327323594311224 ) ) ;
#19736=CARTESIAN_POINT ( 'NONE',  ( -97.09054081448391571, -281.1699180687517696, -225.2831583572297234 ) ) ;
#19737=CARTESIAN_POINT ( 'NONE',  ( -45.92068160576775426, -156.1269989744705526, -363.0336626541780447 ) ) ;
#19738=CARTESIAN_POINT ( 'NONE',  ( 37.84251794672265845, -280.2996511457330939, -284.0696689086099127 ) ) ;
#19739=CARTESIAN_POINT ( 'NONE',  ( -107.0931480392117976, -282.9193594679904891, -243.7795018716523430 ) ) ;
#19740=CARTESIAN_POINT ( 'NONE',  ( -92.93686599548415472, -299.0284833316845834, -218.4851962741639113 ) ) ;
#19741=CARTESIAN_POINT ( 'NONE',  ( 29.90993719255589767, -293.6599345157313223, -241.6799036520421566 ) ) ;
#19743=CARTESIAN_POINT ( 'NONE',  ( -97.15301100410968616, -289.8306929644076604, -227.5684999561558470 ) ) ;
#19744=CARTESIAN_POINT ( 'NONE',  ( -38.53504745781614815, -277.7181572635600446, -347.2499254203794408 ) ) ;
#19745=CARTESIAN_POINT ( 'NONE',  ( -110.3417001280813707, -272.5521521680024648, -270.3611179825603585 ) ) ;
#19747=CARTESIAN_POINT ( 'NONE',  ( -60.76358233746753257, -272.6756696795112020, -197.2789531441635802 ) ) ;
#19751=CARTESIAN_POINT ( 'NONE',  ( 129.4467878515196162, -299.5541904835127980, -198.3997165823495550 ) ) ;
#19752=CARTESIAN_POINT ( 'NONE',  ( -10.85129343070491892, -283.7782516955888354, -338.7705037227991056 ) ) ;
#19753=CARTESIAN_POINT ( 'NONE',  ( 25.43068128015184470, -282.7389056369913760, -227.4487645885667746 ) ) ;
#19754=CARTESIAN_POINT ( 'NONE',  ( -108.3242324399501229, -283.3737599452003906, -288.3857831769414020 ) ) ;
#19755=CARTESIAN_POINT ( 'NONE',  ( -32.91259614913970211, -281.9689674292251880, -196.2581590718765767 ) ) ;
#19756=CARTESIAN_POINT ( 'NONE',  ( 17.02974745033863968, -274.7391166311875850, -320.1238118355374809 ) ) ;
#19758=CARTESIAN_POINT ( 'NONE',  ( 36.00835036207486439, -276.6477944451348776, -271.5764282949344306 ) ) ;
#19760=CARTESIAN_POINT ( 'NONE',  ( -99.51307849737928279, -278.7543702694639478, -315.5374298997721780 ) ) ;
#19764=CARTESIAN_POINT ( 'NONE',  ( -68.02263366361404451, -287.5140618410572415, -201.0722573994112281 ) ) ;
#19765=CARTESIAN_POINT ( 'NONE',  ( 12.45731938454958332, -293.5344078923220650, -324.0277401862096553 ) ) ;
#19766=CARTESIAN_POINT ( 'NONE',  ( -6.967832638906750198, -288.0125230783871757, -341.0205149338335104 ) ) ;
#19767=CARTESIAN_POINT ( 'NONE',  ( -90.37349702975336641, -283.5291129654755196, -218.6581220524021205 ) ) ;
#19768=CARTESIAN_POINT ( 'NONE',  ( -106.7353939726693426, -282.8017453815176623, -295.0056244869351758 ) ) ;
#19769=CARTESIAN_POINT ( 'NONE',  ( -18.23320475851627620, -287.0425047312920128, -341.9185511184355164 ) ) ;
#19770=CARTESIAN_POINT ( 'NONE',  ( -89.16383424396659052, -285.0059014523712904, -322.4093275085817822 ) ) ;
#19771=CARTESIAN_POINT ( 'NONE',  ( 37.70584845660003737, -273.5624502577534827, -271.1760116059775214 ) ) ;
#19772=CARTESIAN_POINT ( 'NONE',  ( 35.09498239607010817, -285.6494295133321089, -246.5412806311888403 ) ) ;
#19773=CARTESIAN_POINT ( 'NONE',  ( -10.04654659474507916, -300.3939934521641248, -195.3518037847966866 ) ) ;
#19774=CARTESIAN_POINT ( 'NONE',  ( -46.26204850434202598, -283.9390585778286322, -195.7256317173185778 ) ) ;
#19775=CARTESIAN_POINT ( 'NONE',  ( -11.67186913108536217, -281.3359232788729400, -201.7183662783044724 ) ) ;
#19776=CARTESIAN_POINT ( 'NONE',  ( 27.33943558787691686, -290.0633536414809441, -308.6544477817870415 ) ) ;
#19779=CARTESIAN_POINT ( 'NONE',  ( -44.63188582019119366, -297.0637387576827564, -345.6210205169334131 ) ) ;
#19781=CARTESIAN_POINT ( 'NONE',  ( -88.88717499401114708, -277.3284010007266716, -215.8094222756787985 ) ) ;
#19782=CARTESIAN_POINT ( 'NONE',  ( -84.15985010224790130, -290.6243338587401013, -209.3660776980017886 ) ) ;
#19783=CARTESIAN_POINT ( 'NONE',  ( 12.88457774571210557, -292.7372404654198590, -324.5029587064720999 ) ) ;
#19784=CARTESIAN_POINT ( 'NONE',  ( -93.45596567768583895, -277.9071474005312439, -222.8819648695211129 ) ) ;
#19785=CARTESIAN_POINT ( 'NONE',  ( -36.44134323252146856, -296.2031237266695598, -196.1261993992958423 ) ) ;
#19786=CARTESIAN_POINT ( 'NONE',  ( 27.60164628934830944, -295.3341227589655205, -304.8734753598757266 ) ) ;
#19787=CARTESIAN_POINT ( 'NONE',  ( 21.31550574532285580, -296.6948066931273615, -317.0979686699210447 ) ) ;
#19788=CARTESIAN_POINT ( 'NONE',  ( -109.1914579710964688, -295.3593595955787805, -244.6644246220234891 ) ) ;
#19790=CARTESIAN_POINT ( 'NONE',  ( 18.68388157314336340, -291.0843738005387422, -219.0278129147083916 ) ) ;
#19792=CARTESIAN_POINT ( 'NONE',  ( -82.10171122319502501, -292.8537390999568402, -211.8850126452549603 ) ) ;
#19794=CARTESIAN_POINT ( 'NONE',  ( -99.85487640567964718, -291.8773005092447761, -232.3518491338498109 ) ) ;
#19795=CARTESIAN_POINT ( 'NONE',  ( 133.0872704186301405, -299.5541904835127980, -201.5153591320744226 ) ) ;
#19796=CARTESIAN_POINT ( 'NONE',  ( -92.53669015439579937, -292.4888117153999474, -217.1676380539473143 ) ) ;
#19797=CARTESIAN_POINT ( 'NONE',  ( 22.08979908418054805, -280.2049567537261510, -316.7101787175686809 ) ) ;
#19798=CARTESIAN_POINT ( 'NONE',  ( 32.62907988878000509, -293.2746562634193310, -249.3761161526255705 ) ) ;
#19799=CARTESIAN_POINT ( 'NONE',  ( 38.25468745361011713, -281.3691200323804651, -255.7260168691857700 ) ) ;
#19801=CARTESIAN_POINT ( 'NONE',  ( -74.26957379479510735, -283.1956220999660445, -337.9637400062198367 ) ) ;
#19802=CARTESIAN_POINT ( 'NONE',  ( -45.58917951545137015, -287.1567656722282322, -344.7385843906310470 ) ) ;
#19803=CARTESIAN_POINT ( 'NONE',  ( -21.14134750837864374, -280.9818320128409255, -342.8599463161110066 ) ) ;
#19804=CARTESIAN_POINT ( 'NONE',  ( -22.68025812134403196, -278.7162612770173951, -195.4224380181877052 ) ) ;
#19805=CARTESIAN_POINT ( 'NONE',  ( -1.103432937216531462, -285.4419472342749486, -202.7720619055572229 ) ) ;
#19807=CARTESIAN_POINT ( 'NONE',  ( 31.56818299172082476, -294.8032841239700019, -243.9439186182547417 ) ) ;
#19808=CARTESIAN_POINT ( 'NONE',  ( 22.28705372150622566, -276.3322010358536431, -222.5594381705689955 ) ) ;
#19809=CARTESIAN_POINT ( 'NONE',  ( -78.64745811923552310, -277.2919877065582455, -330.6383188499635821 ) ) ;
#19810=CARTESIAN_POINT ( 'NONE',  ( -109.8648345067316967, -290.3904830862032895, -296.3918474323584178 ) ) ;
#19811=CARTESIAN_POINT ( 'NONE',  ( -85.20936181462374748, -281.7872532658637965, -328.8247918306738597 ) ) ;
#19813=CARTESIAN_POINT ( 'NONE',  ( 20.70238336388817402, -293.2376174111251999, -315.0391521586855106 ) ) ;
#19814=CARTESIAN_POINT ( 'NONE',  ( -99.86788536775441116, -295.1116386565533389, -228.9194289742398212 ) ) ;
#19817=CARTESIAN_POINT ( 'NONE',  ( -44.29982926479985395, -291.4695650077200071, -197.5808075477365833 ) ) ;
#19818=DIRECTION ( 'NONE',  ( 0.000000000000000000, 0.000000000000000000, -1.000000000000000000 ) ) ;
#19819=CARTESIAN_POINT ( 'NONE',  ( -67.74223827176246004, -280.9809262143061233, -333.4151289067050357 ) ) ;
#19820=CARTESIAN_POINT ( 'NONE',  ( -112.9741625675555809, -295.4423467957212210, -283.7976215715974604 ) ) ;
#19821=CARTESIAN_POINT ( 'NONE',  ( 38.29441365000484154, -279.7583168382161602, -275.5994865863074779 ) ) ;
#19822=CARTESIAN_POINT ( 'NONE',  ( 11.74824306526563511, -288.0322077725974736, -211.6108641715086378 ) ) ;
#19823=CARTESIAN_POINT ( 'NONE',  ( 30.97534841185867549, -287.0404763278103246, -244.4933101193268499 ) ) ;
#19824=CARTESIAN_POINT ( 'NONE',  ( -35.07711795261460708, -278.5433253358024217, -344.0196505608382722 ) ) ;
#19825=CARTESIAN_POINT ( 'NONE',  ( -110.0741409595411255, -294.7888458145322943, -253.5730609785514105 ) ) ;
#19826=CARTESIAN_POINT ( 'NONE',  ( -106.9324130441769398, -297.9793987867762439, -295.7130125659959958 ) ) ;
#19827=CARTESIAN_POINT ( 'NONE',  ( -109.5198074835607258, -277.5218494093459753, -257.0400322831028461 ) ) ;
#19830=CARTESIAN_POINT ( 'NONE',  ( -113.6322613052279706, -296.0854973759957147, -281.0227273243137347 ) ) ;
#19831=CARTESIAN_POINT ( 'NONE',  ( -100.0417524746999050, -291.9279981651594085, -310.4861430031413647 ) ) ;
#19832=CARTESIAN_POINT ( 'NONE',  ( 202.7117753844581500, 291.9766168559941661, -53.99999999997706368 ) ) ;
#19833=CARTESIAN_POINT ( 'NONE',  ( -21.09863385626011123, -289.4896033134440927, -341.6356258090864912 ) ) ;
#19835=CARTESIAN_POINT ( 'NONE',  ( 21.79712709136077109, -279.9509789798811994, -221.4180967335175865 ) ) ;
#19836=CARTESIAN_POINT ( 'NONE',  ( -97.32270926352100560, -296.5577274728772750, -318.5025463817614764 ) ) ;
#19837=CARTESIAN_POINT ( 'NONE',  ( -87.80879734104286172, -289.4951983790995200, -213.8511403055622395 ) ) ;
#19838=CARTESIAN_POINT ( 'NONE',  ( -97.33253926625397412, -297.5320688180210027, -222.1237516451573129 ) ) ;
#19839=CARTESIAN_POINT ( 'NONE',  ( 33.32759624862482895, -293.6428072252660968, -251.9780269348134709 ) ) ;
#19842=CARTESIAN_POINT ( 'NONE',  ( 20.97180904886876718, -289.7413038712097091, -319.5773998617260077 ) ) ;
#19843=CARTESIAN_POINT ( 'NONE',  ( -2.602324593224680793, -279.1233781216987495, -342.4248175857292154 ) ) ;
#19844=VERTEX_POINT ( 'NONE', #69486 ) ;
#19845=CARTESIAN_POINT ( 'NONE',  ( 37.23443169202002423, -280.6657830660437867, -251.6070957540618735 ) ) ;
#19846=CARTESIAN_POINT ( 'NONE',  ( -111.2354060202307977, -286.7054854840063172, -258.4582456560783044 ) ) ;
#19847=CARTESIAN_POINT ( 'NONE',  ( 38.09030551851898849, -286.2845723372089424, -282.8732652393977673 ) ) ;
#19848=CARTESIAN_POINT ( 'NONE',  ( -75.17890104189361011, -271.5469468727137610, -205.7381509177145915 ) ) ;
#19849=CARTESIAN_POINT ( 'NONE',  ( -72.61116682373119602, -275.5019396621260626, -204.7492781176285348 ) ) ;
#19850=CARTESIAN_POINT ( 'NONE',  ( -96.23902366933627661, -289.2605802766945544, -224.8372837746817083 ) ) ;
#19851=CARTESIAN_POINT ( 'NONE',  ( -112.9791290467273654, -280.4683850981388673, -265.9696689317390792 ) ) ;
#19853=CARTESIAN_POINT ( 'NONE',  ( 17.96452820155933594, -280.8733720385426977, -222.6950921471296283 ) ) ;
#19854=CARTESIAN_POINT ( 'NONE',  ( 19.76083203576745362, -280.2568332731972305, -224.7191034666850271 ) ) ;
#19855=CARTESIAN_POINT ( 'NONE',  ( -22.98323590571796160, -277.9524078404988927, -345.7498532214596025 ) ) ;
#19856=CARTESIAN_POINT ( 'NONE',  ( -113.9878542064895584, -277.3316714146322397, -271.5866485534946264 ) ) ;
#19857=CARTESIAN_POINT ( 'NONE',  ( -14.28501004054799317, -91.24624836385295623, -357.5043840972602425 ) ) ;
#19858=CARTESIAN_POINT ( 'NONE',  ( -113.6301709903047339, -273.6005026173463648, -261.8235875350928268 ) ) ;
#19860=CARTESIAN_POINT ( 'NONE',  ( -113.4905809247468369, -274.1437518858514295, -264.6971630283529180 ) ) ;
#19861=CARTESIAN_POINT ( 'NONE',  ( -20.25526795762937127, -282.7662352645560304, -195.3538533559490702 ) ) ;
#19862=CARTESIAN_POINT ( 'NONE',  ( 82.63534306898570492, -300.6190880219792234, -193.0924700335917237 ) ) ;
#19864=CARTESIAN_POINT ( 'NONE',  ( 29.08426838874779108, -288.2148083501572273, -239.3479469218989664 ) ) ;
#19865=CARTESIAN_POINT ( 'NONE',  ( 25.03291158125579585, -289.8944386141885161, -313.8494441673540791 ) ) ;
#19866=CARTESIAN_POINT ( 'NONE',  ( -110.3469302561202454, -289.9618618412728779, -265.7208929794977053 ) ) ;
#19867=CARTESIAN_POINT ( 'NONE',  ( -79.13156295577935850, -283.1074802814790701, -334.9609188179333614 ) ) ;
#19868=CARTESIAN_POINT ( 'NONE',  ( 34.23643778570506413, -279.7168000767629792, -252.3372213726389077 ) ) ;
#19869=CARTESIAN_POINT ( 'NONE',  ( 20.46231358632398312, -288.7647177333050763, -223.7624331235648754 ) ) ;
#19870=CARTESIAN_POINT ( 'NONE',  ( 32.64108156036306241, -279.7265045949353066, -247.1108045521797578 ) ) ;
#19871=CARTESIAN_POINT ( 'NONE',  ( -85.82196974150400592, -280.6790745625722252, -215.1261025035766465 ) ) ;
#19872=CARTESIAN_POINT ( 'NONE',  ( -64.35006221551422811, -277.9065828417870421, -338.3010481819119946 ) ) ;
#19873=CARTESIAN_POINT ( 'NONE',  ( -45.99623230670244567, -287.9543732541552572, -346.5264392340654354 ) ) ;
#19874=CARTESIAN_POINT ( 'NONE',  ( -2.955911128589296499, -283.4122504978410575, -339.0909240032391949 ) ) ;
#19875=CARTESIAN_POINT ( 'NONE',  ( -112.3011926466277828, -285.2615055784484639, -253.0232581102962968 ) ) ;
#19876=CARTESIAN_POINT ( 'NONE',  ( -4.825256163146140587, -282.7781737388872330, -335.7192152346252669 ) ) ;
#19879=CARTESIAN_POINT ( 'NONE',  ( -109.2659381197514961, -292.7191060495488273, -246.3806185591135431 ) ) ;
#19880=CARTESIAN_POINT ( 'NONE',  ( -74.42510646798821483, -290.2543600667134456, -203.4423668922552793 ) ) ;
#19881=CARTESIAN_POINT ( 'NONE',  ( 26.84851775130295692, -274.1296048084064978, -234.9988425568830905 ) ) ;
#19882=CARTESIAN_POINT ( 'NONE',  ( -0.7619821634719919912, -293.9279871557318415, -338.0164812317882479 ) ) ;
#19883=CARTESIAN_POINT ( 'NONE',  ( -99.43629866134806150, -288.4882768012640213, -310.0469918551870023 ) ) ;
#19884=CARTESIAN_POINT ( 'NONE',  ( 30.40877048175368103, -292.1873985034024486, -300.1578920226834271 ) ) ;
#19885=CARTESIAN_POINT ( 'NONE',  ( -108.1045342987575850, -291.4989204700930259, -290.0354864268057895 ) ) ;
#19887=CARTESIAN_POINT ( 'NONE',  ( -100.6003028256002665, -292.0089555232320322, -310.7474559801054284 ) ) ;
#19888=CARTESIAN_POINT ( 'NONE',  ( -11.75283257161107109, -290.3842436657230337, -199.6294066718878639 ) ) ;
#19889=CARTESIAN_POINT ( 'NONE',  ( -43.67058894805948199, -297.1322664049901050, -345.1064105123521131 ) ) ;
#19890=CARTESIAN_POINT ( 'NONE',  ( -14.50397283338986121, -287.2967096829185039, -200.7245528512789292 ) ) ;
#19891=CARTESIAN_POINT ( 'NONE',  ( 33.76072934726541064, -295.8689257727005497, -294.9025961025897118 ) ) ;
#19892=CARTESIAN_POINT ( 'NONE',  ( 23.14423652758372540, -276.9213866659573569, -225.4182846009512957 ) ) ;
#19893=CARTESIAN_POINT ( 'NONE',  ( -113.4421986318000535, -272.0436218923558158, -258.9516208099599908 ) ) ;
#19894=CARTESIAN_POINT ( 'NONE',  ( 16.31731558162838169, -274.5168461903443244, -321.3384075001269480 ) ) ;
#19895=CARTESIAN_POINT ( 'NONE',  ( -2.452958930701184315, -278.5972204303146782, -204.5888456860378426 ) ) ;
#19896=CARTESIAN_POINT ( 'NONE',  ( -85.58263452931861082, -274.5725946120732033, -214.9766168087108156 ) ) ;
#19897=CARTESIAN_POINT ( 'NONE',  ( 4.555368497081262014, -273.1799583960502673, -206.3980818031283775 ) ) ;
#19898=CARTESIAN_POINT ( 'NONE',  ( -108.4093961080431683, -298.2282379495194959, -251.2138890455044020 ) ) ;
#19900=CARTESIAN_POINT ( 'NONE',  ( -110.5360380290351685, -297.3763345195026773, -268.7394961063603773 ) ) ;
#19902=CARTESIAN_POINT ( 'NONE',  ( 36.67934959249920723, -285.3918560906939206, -256.2440714191681082 ) ) ;
#19903=CARTESIAN_POINT ( 'NONE',  ( -36.48340605792428448, -298.0631913788034240, -197.3611179848009272 ) ) ;
#19904=CARTESIAN_POINT ( 'NONE',  ( -64.54719059175596385, -285.7066592465739063, -198.3131993125137740 ) ) ;
#19905=CARTESIAN_POINT ( 'NONE',  ( -40.34218509302081657, -288.7555934237355473, -347.2945534490193609 ) ) ;
#19906=CARTESIAN_POINT ( 'NONE',  ( -112.4828589344016621, -298.6129001573509640, -264.0342027524442869 ) ) ;
#19907=CARTESIAN_POINT ( 'NONE',  ( 11.46853091089890953, -292.3731666252827495, -327.0849204777914565 ) ) ;
#19909=CARTESIAN_POINT ( 'NONE',  ( 20.95029152622550939, -280.0720102686328232, -220.2791208003248471 ) ) ;
#19911=CARTESIAN_POINT ( 'NONE',  ( -4.829096099716524648, -286.1237833571632905, -337.9475929042657754 ) ) ;
#19912=CARTESIAN_POINT ( 'NONE',  ( -56.64738604829841506, -277.8032505011321405, -197.8352665249953759 ) ) ;
#19913=CARTESIAN_POINT ( 'NONE',  ( 1.508823052283176480, -287.3150962168544993, -332.6328399207702660 ) ) ;
#19914=LINE ( 'NONE', #63510, #41124 ) ;
#19915=CARTESIAN_POINT ( 'NONE',  ( -7.444013132586889014, -286.6601309731845504, -339.1998302859839214 ) ) ;
#19916=CARTESIAN_POINT ( 'NONE',  ( -103.8389552304829806, -274.4977754644102674, -238.5991467853361314 ) ) ;
#19917=CARTESIAN_POINT ( 'NONE',  ( -111.0333716389159520, -270.8448262217655724, -253.6622631491634081 ) ) ;
#19918=CARTESIAN_POINT ( 'NONE',  ( 34.23067989249568654, -281.7424991422525977, -284.7904588454235864 ) ) ;
#19919=CARTESIAN_POINT ( 'NONE',  ( -98.23527737376741698, -297.3482087257295348, -223.2126454528674060 ) ) ;
#19920=CARTESIAN_POINT ( 'NONE',  ( 21.13882259146600973, -276.3539895397269675, -225.6704442333011116 ) ) ;
#19921=CARTESIAN_POINT ( 'NONE',  ( 37.55129286434630842, -285.5043265248769444, -260.3434436863306587 ) ) ;
#19922=CARTESIAN_POINT ( 'NONE',  ( 0.3463326565518302647, -282.5539307346783175, -205.4590133269092007 ) ) ;
#19923=CARTESIAN_POINT ( 'NONE',  ( -34.45629250580390135, -297.1478904710399433, -197.1262973527614122 ) ) ;
#19928=CARTESIAN_POINT ( 'NONE',  ( -111.9541447851175917, -286.5604026035442757, -268.1634141801937403 ) ) ;
#19930=CARTESIAN_POINT ( 'NONE',  ( -72.02372285203398405, -277.1237833571632905, -198.2697987213421698 ) ) ;
#19931=CARTESIAN_POINT ( 'NONE',  ( 36.72722915942244981, -275.0065250947175741, -290.8540413367579163 ) ) ;
#19933=CARTESIAN_POINT ( 'NONE',  ( -95.65329390752376071, -285.4435574264955449, -315.4424003221237740 ) ) ;
#19934=CARTESIAN_POINT ( 'NONE',  ( 12.30073783424776401, -277.9478274967066795, -325.0388014569549000 ) ) ;
#19935=CARTESIAN_POINT ( 'NONE',  ( -97.56870268527291046, -285.3442247216904093, -317.3857334328633328 ) ) ;
#19936=CARTESIAN_POINT ( 'NONE',  ( -93.73696302578666462, -282.6841478574131656, -317.3366949206035770 ) ) ;
#19937=CARTESIAN_POINT ( 'NONE',  ( -5.955068411925046767, -282.4648207036316876, -202.2304355248318188 ) ) ;
#19938=CARTESIAN_POINT ( 'NONE',  ( -67.53759791116084443, -273.8334939040555014, -199.5288671246859735 ) ) ;
#19939=CARTESIAN_POINT ( 'NONE',  ( 23.63414251517103537, -274.7577112414791145, -223.3189515870644186 ) ) ;
#19940=CARTESIAN_POINT ( 'NONE',  ( -107.3329321399949379, -298.1393858440949316, -295.8609516453394690 ) ) ;
#19943=CARTESIAN_POINT ( 'NONE',  ( -112.4317632126142428, -294.5586089432812855, -280.8352438237027400 ) ) ;
#19945=CARTESIAN_POINT ( 'NONE',  ( 11.78444874418207355, -275.8556887629201810, -324.5094260177707497 ) ) ;
#19946=CARTESIAN_POINT ( 'NONE',  ( -65.49921320297718808, -287.4391688771809754, -201.8585564823362972 ) ) ;
#19947=CARTESIAN_POINT ( 'NONE',  ( 21.76201296504892468, -295.7261785416021098, -318.6461051238221671 ) ) ;
#19948=CARTESIAN_POINT ( 'NONE',  ( 37.68481274290093097, -294.9515811969549759, -285.8217481897000880 ) ) ;
#19949=CARTESIAN_POINT ( 'NONE',  ( -108.7586984996972888, -292.8417942537846557, -247.9652572111156985 ) ) ;
#19950=CARTESIAN_POINT ( 'NONE',  ( -105.9624606558039943, -276.1589251778424341, -300.3443685384220316 ) ) ;
#19951=CARTESIAN_POINT ( 'NONE',  ( -70.40140500038901905, -281.5330995528415770, -203.6508939139774270 ) ) ;
#19952=CARTESIAN_POINT ( 'NONE',  ( -35.64177008129143331, -293.1105389541633599, -344.7944523728916124 ) ) ;
#19953=CARTESIAN_POINT ( 'NONE',  ( -101.8537276316863540, -285.8847908249632610, -310.0915066855704936 ) ) ;
#19954=CARTESIAN_POINT ( 'NONE',  ( -104.8769846099606582, -283.8551728052002545, -241.7138367005689190 ) ) ;
#19955=CARTESIAN_POINT ( 'NONE',  ( 191.3713445966495499, 269.3054100996118336, -138.9528838864912075 ) ) ;
#19957=CARTESIAN_POINT ( 'NONE',  ( -107.0073016536492503, -283.9289337795021311, -292.2424216654995348 ) ) ;
#19959=CARTESIAN_POINT ( 'NONE',  ( 25.68417001321747506, -283.2116068919356735, -314.0789815084744987 ) ) ;
#19960=CARTESIAN_POINT ( 'NONE',  ( -100.6595828943831492, -283.9196741993933983, -227.1530082133320434 ) ) ;
#19961=CARTESIAN_POINT ( 'NONE',  ( -61.98348121027238022, -280.6808443343365980, -197.6029025719920753 ) ) ;
#19962=CARTESIAN_POINT ( 'NONE',  ( -106.9357426684950241, -279.6674795972777474, -301.7846174024846277 ) ) ;
#19963=CARTESIAN_POINT ( 'NONE',  ( -73.72474628654926221, -280.2335615410636365, -202.5996975595941478 ) ) ;
#19964=CARTESIAN_POINT ( 'NONE',  ( -53.28691492658257545, -271.3380690714491266, -200.3538533559491555 ) ) ;
#19965=CARTESIAN_POINT ( 'NONE',  ( 198.6655289599987384, 284.5870187839926757, -111.8036103090564382 ) ) ;
#19966=CARTESIAN_POINT ( 'NONE',  ( -40.88665857834944717, -276.0077436703259082, -195.5608444318603745 ) ) ;
#19967=CARTESIAN_POINT ( 'NONE',  ( 160.4760655529063911, 220.5667256801315261, -205.0173812340459563 ) ) ;
#19968=CARTESIAN_POINT ( 'NONE',  ( -97.72166288328035932, -277.1729728092930714, -226.4736835347069643 ) ) ;
#19969=CARTESIAN_POINT ( 'NONE',  ( -5.055330749482738639, -294.2315037087241762, -201.5747503673869119 ) ) ;
#19970=CARTESIAN_POINT ( 'NONE',  ( -9.199295319417219119, -294.0228281539394857, -337.8424952510208641 ) ) ;
#19971=CARTESIAN_POINT ( 'NONE',  ( -111.4843484015535324, -289.8021139158824440, -290.9133589880916588 ) ) ;
#19973=CARTESIAN_POINT ( 'NONE',  ( -88.22667549685542099, -294.3226516898990326, -327.4349416818520808 ) ) ;
#19974=CARTESIAN_POINT ( 'NONE',  ( -27.71220996078968568, -284.5763507776962911, -197.1920443709530275 ) ) ;
#19975=CARTESIAN_POINT ( 'NONE',  ( -0.6667090460061715351, -294.4052438684481103, -205.8033098007449269 ) ) ;
#19976=CARTESIAN_POINT ( 'NONE',  ( -14.33130992332623421, -284.8357321918245475, -200.2988074116600501 ) ) ;
#19977=CARTESIAN_POINT ( 'NONE',  ( -110.8027547118739449, -285.8957914225510990, -268.1892671417301699 ) ) ;
#19979=CARTESIAN_POINT ( 'NONE',  ( -88.50161931618738720, -292.2964152334592427, -213.1292834756512775 ) ) ;
#19980=CARTESIAN_POINT ( 'NONE',  ( -61.54920342400573219, -283.8675183020607165, -339.3490416550471878 ) ) ;
#19981=CARTESIAN_POINT ( 'NONE',  ( -53.22199430612302251, -294.0462103635840094, -345.3541904683731332 ) ) ;
#19982=CARTESIAN_POINT ( 'NONE',  ( -107.1180926905573756, -291.7688997321332636, -238.0564648206466245 ) ) ;
#19983=CARTESIAN_POINT ( 'NONE',  ( -103.7421441121441603, -290.5370580429944880, -309.3317350788577187 ) ) ;
#19984=CARTESIAN_POINT ( 'NONE',  ( 34.52206291861869403, -287.8880770959629558, -283.1907541928001137 ) ) ;
#19987=CARTESIAN_POINT ( 'NONE',  ( -111.9827764451988799, -298.2435621634423342, -283.6576445192034726 ) ) ;
#19988=CARTESIAN_POINT ( 'NONE',  ( -98.68692294464464965, -295.8492338798204173, -224.6220641093916868 ) ) ;
#19989=CARTESIAN_POINT ( 'NONE',  ( 22.31209271670305938, -280.0193616749232888, -227.8777865722506135 ) ) ;
#19990=CARTESIAN_POINT ( 'NONE',  ( 37.84419997751617615, -275.2649468118802361, -286.7507640890440257 ) ) ;
#19991=CARTESIAN_POINT ( 'NONE',  ( -103.1427785231897616, -295.4794976754084814, -237.0673529196825484 ) ) ;
#19992=CARTESIAN_POINT ( 'NONE',  ( -97.87948571183410706, -279.8223121641687499, -313.3487764013228798 ) ) ;
#19993=CARTESIAN_POINT ( 'NONE',  ( -4.744646648621247742, -272.6257127552618158, -203.6514982731144698 ) ) ;
#19995=CARTESIAN_POINT ( 'NONE',  ( -31.55582687073997405, -296.1827040247025593, -343.5801729685740042 ) ) ;
#19996=CARTESIAN_POINT ( 'NONE',  ( -108.8905680528670246, -297.4220659071904151, -286.3293856841414708 ) ) ;
#19998=CARTESIAN_POINT ( 'NONE',  ( -32.04753574849496545, -296.5865674671629222, -346.3901031670015414 ) ) ;
#20000=CARTESIAN_POINT ( 'NONE',  ( -72.40225788177887978, -295.5895106912616939, -203.8146963531014251 ) ) ;
#20001=CARTESIAN_POINT ( 'NONE',  ( -6.005447940128382456, -293.1266639701533450, -204.3023939260049247 ) ) ;
#20002=CARTESIAN_POINT ( 'NONE',  ( -55.30580511946723021, -274.6295514870644183, -195.6520171189104360 ) ) ;
#20003=CARTESIAN_POINT ( 'NONE',  ( -106.5931539357383855, -288.7980200035270286, -295.2531058900292464 ) ) ;
#20005=CARTESIAN_POINT ( 'NONE',  ( -104.1791820075805504, -273.5410518952702432, -232.1454206897277288 ) ) ;
#20007=CARTESIAN_POINT ( 'NONE',  ( -75.22524286702045515, -297.8657468433290205, -207.8771396955177693 ) ) ;
#20009=CARTESIAN_POINT ( 'NONE',  ( -14.74552191971798010, -282.3232764346112162, -198.4188702412958776 ) ) ;
#20010=CARTESIAN_POINT ( 'NONE',  ( 37.65877536361002598, -280.4271376863619594, -285.4683000579449867 ) ) ;
#20011=CARTESIAN_POINT ( 'NONE',  ( -31.46634335474100652, -276.3285291766658247, -347.0869588441506721 ) ) ;
#20012=CARTESIAN_POINT ( 'NONE',  ( 19.54517269016981729, -279.2573273944075822, -219.6431280061817972 ) ) ;
#20013=CARTESIAN_POINT ( 'NONE',  ( 29.11317099448432444, -279.0860963724547901, -235.1248985799621778 ) ) ;
#20014=CARTESIAN_POINT ( 'NONE',  ( -57.00171108673121267, -272.3684171248539201, -199.3935320658721650 ) ) ;
#20015=CARTESIAN_POINT ( 'NONE',  ( -97.20430083200136551, -281.1703169608771304, -225.1575159393051138 ) ) ;
#20018=CARTESIAN_POINT ( 'NONE',  ( -92.90624787607011115, -295.5087688527922865, -218.4524048373820335 ) ) ;
#20019=CARTESIAN_POINT ( 'NONE',  ( -4.604144321097812131, -292.4716473784062032, -200.6671265644712037 ) ) ;
#20020=CARTESIAN_POINT ( 'NONE',  ( 35.12510414080808374, -277.8090652632523074, -290.3739080526739826 ) ) ;
#20021=CARTESIAN_POINT ( 'NONE',  ( -33.92475487546162327, -272.0949882399519879, -195.4389908371266245 ) ) ;
#20024=CARTESIAN_POINT ( 'NONE',  ( 22.28199568906610395, -284.1043718082944451, -316.7967854410098312 ) ) ;
#20026=CARTESIAN_POINT ( 'NONE',  ( 0.8551782934694188709, -284.5611025376319958, -205.7571982348605673 ) ) ;
#20028=CARTESIAN_POINT ( 'NONE',  ( 20.82856513173618040, -292.9738363566014527, -315.1404969690702274 ) ) ;
#20029=CARTESIAN_POINT ( 'NONE',  ( 35.21295173079262497, -285.8962048697335376, -286.1269500914702348 ) ) ;
#20031=CARTESIAN_POINT ( 'NONE',  ( 17.60757943251340762, -292.2661600556220378, -321.4059739920773495 ) ) ;
#20032=CARTESIAN_POINT ( 'NONE',  ( -68.20244818725494440, -284.1340704704256268, -200.5591808367052806 ) ) ;
#20033=CARTESIAN_POINT ( 'NONE',  ( -111.0786297607549642, -280.1124829652855510, -273.4116296694433004 ) ) ;
#20034=CARTESIAN_POINT ( 'NONE',  ( 38.28548676386245830, -288.9144956966022733, -282.8715916027106232 ) ) ;
#20035=CARTESIAN_POINT ( 'NONE',  ( 36.99803877511962469, -279.5918201155166116, -254.5641974274557811 ) ) ;
#20036=CARTESIAN_POINT ( 'NONE',  ( 34.01067763643982289, -287.7563193171338298, -285.8417480492505547 ) ) ;
#20037=CARTESIAN_POINT ( 'NONE',  ( -54.64883464035107608, -281.2507713869273971, -198.7834094798326134 ) ) ;
#20038=CARTESIAN_POINT ( 'NONE',  ( -64.88637029251910349, -280.4857530425537107, -202.5828554443387759 ) ) ;
#20039=CARTESIAN_POINT ( 'NONE',  ( -62.67277580053323760, -287.7039761364958395, -199.3911003191245186 ) ) ;
#20041=CARTESIAN_POINT ( 'NONE',  ( -93.66130201641277608, -297.1019729443513029, -217.7752289675644874 ) ) ;
#20042=CARTESIAN_POINT ( 'NONE',  ( -75.53633936148847283, -291.5441692366258053, -334.5089353002856569 ) ) ;
#20044=CARTESIAN_POINT ( 'NONE',  ( -19.11405058567862625, -294.7662352645559736, -190.3538533559490702 ) ) ;
#20046=CARTESIAN_POINT ( 'NONE',  ( -32.76808252924960385, -272.1094782166812251, -195.3208826116317880 ) ) ;
#20048=CARTESIAN_POINT ( 'NONE',  ( -92.13604411657455273, -294.2190398984069475, -323.3141186699876357 ) ) ;
#20049=CARTESIAN_POINT ( 'NONE',  ( -47.27491394963309546, -297.4303200076844291, -197.9267195464555016 ) ) ;
#20050=CARTESIAN_POINT ( 'NONE',  ( 1.695109183097748051, -290.0398546098388692, -332.8657999730142478 ) ) ;
#20051=CARTESIAN_POINT ( 'NONE',  ( 25.99195518158492035, -282.7911378813158763, -231.9627339860960547 ) ) ;
#20052=CARTESIAN_POINT ( 'NONE',  ( -37.48375456549062079, -290.3690268334146936, -346.8808256503987195 ) ) ;
#20053=CARTESIAN_POINT ( 'NONE',  ( -73.35618142252829443, -287.5746980787349685, -204.5592937361379597 ) ) ;
#20054=CARTESIAN_POINT ( 'NONE',  ( -94.96319964996769158, -279.4108287468890239, -219.2850688267585895 ) ) ;
#20055=CARTESIAN_POINT ( 'NONE',  ( -32.13658348927195618, -293.0668532447227790, -345.7546324691795121 ) ) ;
#20056=CARTESIAN_POINT ( 'NONE',  ( 27.85248385341587252, -280.8478708096207583, -229.2890245579890802 ) ) ;
#20057=CARTESIAN_POINT ( 'NONE',  ( 34.04130678602621174, -277.1454403860069533, -249.7979589964799061 ) ) ;
#20058=CARTESIAN_POINT ( 'NONE',  ( 27.33386217378599881, -277.6233781216988064, -239.1787733560258573 ) ) ;
#20059=CARTESIAN_POINT ( 'NONE',  ( 38.12837484848169822, -273.9096893195509779, -279.6466119788075275 ) ) ;
#20062=CARTESIAN_POINT ( 'NONE',  ( 32.79542189131238672, -280.7893188386312886, -249.8971849152191851 ) ) ;
#20064=CARTESIAN_POINT ( 'NONE',  ( -68.83801591382037088, -278.6621530774514213, -340.2037419698561393 ) ) ;
#20065=CARTESIAN_POINT ( 'NONE',  ( -64.76827231773779658, -275.0015256347070931, -202.1637746357501726 ) ) ;
#20066=CARTESIAN_POINT ( 'NONE',  ( -113.5845479338653519, -283.7229996255427409, -261.4253264038227940 ) ) ;
#20067=CARTESIAN_POINT ( 'NONE',  ( -95.09552022463829246, -292.9576642491689427, -224.0541454722773267 ) ) ;
#20068=CARTESIAN_POINT ( 'NONE',  ( -93.56886751066616625, -274.8592502623891392, -218.9128074112863658 ) ) ;
#20070=CARTESIAN_POINT ( 'NONE',  ( -36.95912481475801314, -275.3720476784394009, -193.8422551742366693 ) ) ;
#20072=CARTESIAN_POINT ( 'NONE',  ( -21.65509044688186435, -276.6788735553477636, -341.7077821993584053 ) ) ;
#20073=CARTESIAN_POINT ( 'NONE',  ( -91.72241644707095531, -297.8292329130355256, -321.8435559369090129 ) ) ;
#20074=CARTESIAN_POINT ( 'NONE',  ( -82.56679668817990603, -283.4324854685679611, -210.7396531851886152 ) ) ;
#20076=CARTESIAN_POINT ( 'NONE',  ( -36.37436963039452564, -291.7306902225533918, -193.3753110228519461 ) ) ;
#20077=CARTESIAN_POINT ( 'NONE',  ( 29.49220761520184553, -274.0144666445947905, -303.7202385540210798 ) ) ;
#20078=CARTESIAN_POINT ( 'NONE',  ( -5.937388334416650260, -290.2463030297726050, -339.7888474456598260 ) ) ;
#20079=CARTESIAN_POINT ( 'NONE',  ( -110.6462937780810307, -289.4617814156164286, -271.1751342254810879 ) ) ;
#20081=CARTESIAN_POINT ( 'NONE',  ( -33.55030903467089587, -290.6737327303923166, -194.0444641822093388 ) ) ;
#20082=CARTESIAN_POINT ( 'NONE',  ( -86.74680755776698504, -289.4284379574972945, -324.1998089338482032 ) ) ;
#20084=CARTESIAN_POINT ( 'NONE',  ( 20.04626073632925198, -287.9391673013628861, -219.4092285710269152 ) ) ;
#20085=CARTESIAN_POINT ( 'NONE',  ( -108.9088177157139796, -279.0774796836156497, -255.7988221804640148 ) ) ;
#20086=CARTESIAN_POINT ( 'NONE',  ( -98.03827912585100535, -294.8442727680667304, -317.2377412505912275 ) ) ;
#20087=CARTESIAN_POINT ( 'NONE',  ( -97.50584265687383834, -285.8455798200195090, -222.4696913907785074 ) ) ;
#20088=CARTESIAN_POINT ( 'NONE',  ( -100.9814059380279474, -285.4577828819154206, -226.9572253947787033 ) ) ;
#20089=CARTESIAN_POINT ( 'NONE',  ( 33.34504874474222902, -282.1277551011364153, -288.7268030233975082 ) ) ;
#20090=CARTESIAN_POINT ( 'NONE',  ( 185.2826429462496947, 263.6716433825772583, -153.3442153897663616 ) ) ;
#20091=CARTESIAN_POINT ( 'NONE',  ( 159.7575371838252920, 220.4114972407526523, -204.4531022271711720 ) ) ;
#20092=CARTESIAN_POINT ( 'NONE',  ( 152.4322389789791998, 205.2264399568286706, -214.4046794774016576 ) ) ;
#20093=CARTESIAN_POINT ( 'NONE',  ( 9.596493148575063969, -273.9141057013902127, -214.1751838174417628 ) ) ;
#20094=CARTESIAN_POINT ( 'NONE',  ( -21.85538011468237229, -273.1756386990497276, -198.7063905385278133 ) ) ;
#20095=CARTESIAN_POINT ( 'NONE',  ( -110.2893569753809402, -295.7515852926684374, -294.8185557810772934 ) ) ;
#20096=CARTESIAN_POINT ( 'NONE',  ( 139.6181910892751716, 178.0063059127244856, -238.5957382375125064 ) ) ;
#20097=CARTESIAN_POINT ( 'NONE',  ( 37.15855946076516148, -274.0172280141567853, -252.8969037922039149 ) ) ;
#20098=CARTESIAN_POINT ( 'NONE',  ( -63.53714435172094710, -299.5676532963165073, -200.8469228458471605 ) ) ;
#20099=CARTESIAN_POINT ( 'NONE',  ( -17.36149982982482953, -293.3956680683000400, -199.7745010282513647 ) ) ;
#20101=CARTESIAN_POINT ( 'NONE',  ( -110.5922287740041554, -297.7847741135059323, -247.2244140488346602 ) ) ;
#20102=CARTESIAN_POINT ( 'NONE',  ( -8.188177821665913569, -289.1522358358262750, -337.4081945741010600 ) ) ;
#20104=CARTESIAN_POINT ( 'NONE',  ( -113.2316824492032765, -297.5068725265143144, -258.2415258761737391 ) ) ;
#20105=CARTESIAN_POINT ( 'NONE',  ( -56.04924808363270472, -295.7792095461983308, -344.9905662757627169 ) ) ;
#20106=CARTESIAN_POINT ( 'NONE',  ( -22.74270262261855180, -292.4109186769933331, -198.8358128359274133 ) ) ;
#20109=CARTESIAN_POINT ( 'NONE',  ( 36.77474715412966333, -277.6596393236907829, -285.0603167087974725 ) ) ;
#20110=VERTEX_POINT ( 'NONE', #35838 ) ;
#20111=CARTESIAN_POINT ( 'NONE',  ( 10.78940024551518562, -280.2047063490701362, -210.2684645879271841 ) ) ;
#20112=CARTESIAN_POINT ( 'NONE',  ( 15.77676739851996501, -277.2178036085222743, -320.7777507121354006 ) ) ;
#20113=CARTESIAN_POINT ( 'NONE',  ( 33.76550065166610892, -276.9688174047132634, -243.5704477892614648 ) ) ;
#20114=CARTESIAN_POINT ( 'NONE',  ( -37.15686973064618570, -275.0699269267319664, -345.7288748229163957 ) ) ;
#20115=CARTESIAN_POINT ( 'NONE',  ( -37.83151420578207791, -298.6972715054471337, -197.2608255704180920 ) ) ;
#20116=CARTESIAN_POINT ( 'NONE',  ( -109.3519788511818263, -295.3260676909511062, -255.1383242376388694 ) ) ;
#20117=CARTESIAN_POINT ( 'NONE',  ( -100.4114633486748858, -278.4615197745321211, -314.4262047359401890 ) ) ;
#20118=CARTESIAN_POINT ( 'NONE',  ( -29.71131375633569505, -277.1196749686742464, -343.0121425007147309 ) ) ;
#20119=CARTESIAN_POINT ( 'NONE',  ( 1.287239695076142443, -285.2416008112440977, -204.3072262123218366 ) ) ;
#20120=CARTESIAN_POINT ( 'NONE',  ( -112.3426463542470799, -274.5878523713495838, -267.5935413054058927 ) ) ;
#20121=CARTESIAN_POINT ( 'NONE',  ( 82.61849213892784860, -301.9425569738761510, -196.1180017367229880 ) ) ;
#20123=CARTESIAN_POINT ( 'NONE',  ( 25.83032970961048846, -287.2559421351874676, -307.3651295578798113 ) ) ;
#20125=CARTESIAN_POINT ( 'NONE',  ( -27.40037784261229703, -278.4198998218683982, -196.9665660256600006 ) ) ;
#20126=CARTESIAN_POINT ( 'NONE',  ( -54.61361778231162845, -278.4006854406470666, -198.7749040549008441 ) ) ;
#20127=CARTESIAN_POINT ( 'NONE',  ( -101.6573424560296957, -282.1275674972855541, -307.8419443853190955 ) ) ;
#20128=CARTESIAN_POINT ( 'NONE',  ( -38.77567384759880298, -288.0343566558874500, -195.3621995646847154 ) ) ;
#20129=CARTESIAN_POINT ( 'NONE',  ( 24.32629861042931552, -277.3063535309164536, -310.2567247996188939 ) ) ;
#20132=CARTESIAN_POINT ( 'NONE',  ( -93.23819352308036912, -293.2486548172820449, -220.3552915587440566 ) ) ;
#20133=CARTESIAN_POINT ( 'NONE',  ( -28.73832709560946697, -275.1844852894727183, -345.9120399221340563 ) ) ;
#20135=CARTESIAN_POINT ( 'NONE',  ( 15.67751261981096000, -276.9280115873633576, -320.6886029962282123 ) ) ;
#20136=CARTESIAN_POINT ( 'NONE',  ( 35.42360950894337179, -283.7939573953727859, -289.2088802653337325 ) ) ;
#20139=CARTESIAN_POINT ( 'NONE',  ( -20.78761857074142938, -290.7615670060641264, -344.1390953996880739 ) ) ;
#20141=CARTESIAN_POINT ( 'NONE',  ( -17.69740863898349303, -292.7987519615044789, -342.7959879880374388 ) ) ;
#20143=CARTESIAN_POINT ( 'NONE',  ( 25.70745865827042920, -273.7198733116884455, -232.4994721079409317 ) ) ;
#20144=CARTESIAN_POINT ( 'NONE',  ( 17.66919031077154045, -290.9887443108297020, -220.4392572792103806 ) ) ;
#20147=CARTESIAN_POINT ( 'NONE',  ( -40.58341442781975417, -290.4919935937610376, -194.1102747254016094 ) ) ;
#20148=CARTESIAN_POINT ( 'NONE',  ( 36.83084173599346656, -286.0019373028050040, -286.9252314698308055 ) ) ;
#20151=CARTESIAN_POINT ( 'NONE',  ( -104.6449366095063027, -285.5801239586100451, -300.1209781073677050 ) ) ;
#20152=CARTESIAN_POINT ( 'NONE',  ( -85.84082221598471563, -286.1631219849281820, -215.5171537372244472 ) ) ;
#20153=CARTESIAN_POINT ( 'NONE',  ( -47.54616045868586838, -293.9030850245948159, -195.6473976999308206 ) ) ;
#20154=CARTESIAN_POINT ( 'NONE',  ( 33.83608930054545993, -273.9599221947258911, -295.8733605699800364 ) ) ;
#20155=CARTESIAN_POINT ( 'NONE',  ( 31.22953744634706652, -275.4347737680809018, -235.3792702762425506 ) ) ;
#20157=CARTESIAN_POINT ( 'NONE',  ( -111.2266390754934946, -288.8343882334787054, -254.4783484646853537 ) ) ;
#20158=CARTESIAN_POINT ( 'NONE',  ( -7.884636678422499045, -276.6767267706535449, -341.5180861090478857 ) ) ;
#20159=CARTESIAN_POINT ( 'NONE',  ( -105.4267562159298137, -298.1274605023674553, -301.0859327147970816 ) ) ;
#20162=CARTESIAN_POINT ( 'NONE',  ( -110.5886280708645160, -283.1582098256154154, -276.3720267395096357 ) ) ;
#20163=CARTESIAN_POINT ( 'NONE',  ( -53.30917782360364043, -277.8473460191802360, -197.0274110760031760 ) ) ;
#20164=CARTESIAN_POINT ( 'NONE',  ( -2.853431178006288871, -272.9794744330255867, -202.2784400007492422 ) ) ;
#20165=CARTESIAN_POINT ( 'NONE',  ( -109.3879580793719413, -277.7366946234744205, -282.8137408938397357 ) ) ;
#20166=CARTESIAN_POINT ( 'NONE',  ( -26.08256051640834983, -296.4263249035763579, -343.1892686268481043 ) ) ;
#20168=CARTESIAN_POINT ( 'NONE',  ( -40.97992034744468981, -278.9277414701869588, -193.7434333128720993 ) ) ;
#20169=CARTESIAN_POINT ( 'NONE',  ( -55.85123976163615822, -296.2374980330741323, -341.2713093379865654 ) ) ;
#20170=CARTESIAN_POINT ( 'NONE',  ( -0.9260546494287595909, -295.8942566626101325, -337.6603729592434888 ) ) ;
#20171=CARTESIAN_POINT ( 'NONE',  ( -102.0472147585561515, -272.6806025721981541, -236.4095710574711404 ) ) ;
#20172=CARTESIAN_POINT ( 'NONE',  ( -38.96574107484891414, -294.0319303747026538, -195.3786990875417189 ) ) ;
#20173=CARTESIAN_POINT ( 'NONE',  ( -37.98457500666072661, -286.2109853173925558, -193.3638016889015887 ) ) ;
#20174=CARTESIAN_POINT ( 'NONE',  ( 24.33538729457488614, -273.0991493527042167, -226.3361606592911812 ) ) ;
#20175=CARTESIAN_POINT ( 'NONE',  ( -48.87109260429120638, -289.0283139329745268, -346.5470079670103019 ) ) ;
#20176=CARTESIAN_POINT ( 'NONE',  ( -54.90369035024288991, -281.8053020300051230, -197.7582857938907352 ) ) ;
#20177=CARTESIAN_POINT ( 'NONE',  ( 7.079127850946671963, -285.7325377364758197, -212.0716252673045119 ) ) ;
#20178=CARTESIAN_POINT ( 'NONE',  ( -93.96551828184074395, -287.8695570610788081, -319.5418445805968872 ) ) ;
#20179=CARTESIAN_POINT ( 'NONE',  ( 139.3989977797154154, 177.7276089766264704, -238.0725708408485843 ) ) ;
#20180=CARTESIAN_POINT ( 'NONE',  ( 32.33416872850242640, -286.7681413187816020, -248.3360072627604325 ) ) ;
#20182=CARTESIAN_POINT ( 'NONE',  ( 38.64008698756167348, -282.6305856204697875, -281.2967587790881794 ) ) ;
#20183=CARTESIAN_POINT ( 'NONE',  ( -112.4073492084067851, -289.8131316561925246, -254.2377481203194520 ) ) ;
#20184=CARTESIAN_POINT ( 'NONE',  ( -107.9078311530945058, -279.7832309258712371, -299.1163186579315720 ) ) ;
#20185=CARTESIAN_POINT ( 'NONE',  ( -64.58250098870418299, -281.0191529625151361, -198.8123268789160534 ) ) ;
#20186=CARTESIAN_POINT ( 'NONE',  ( 27.78235261977501835, -280.9363061009318017, -237.2663388890804015 ) ) ;
#20187=CARTESIAN_POINT ( 'NONE',  ( 35.44414798062614835, -277.3199673566674619, -252.2718679261091665 ) ) ;
#20188=CARTESIAN_POINT ( 'NONE',  ( -47.63157325885072879, -295.1795367299789632, -346.6704785548560608 ) ) ;
#20189=CARTESIAN_POINT ( 'NONE',  ( -103.1038996189127346, -288.1000290318023076, -305.7862101314099732 ) ) ;
#20190=CARTESIAN_POINT ( 'NONE',  ( -103.0513045628199649, -295.0323738833450307, -302.9793209375142169 ) ) ;
#20193=CARTESIAN_POINT ( 'NONE',  ( 25.35625050481410625, -284.0177780539782475, -310.5842330859917411 ) ) ;
#20194=CARTESIAN_POINT ( 'NONE',  ( -97.20314257997455343, -295.6359571892910481, -312.1785209911674883 ) ) ;
#20195=AXIS2_PLACEMENT_3D ( 'NONE', #84515, #77431, #69860 ) ;
#20196=CARTESIAN_POINT ( 'NONE',  ( 23.72073476802203018, -294.0107570384902829, -223.9404656963076548 ) ) ;
#20197=CARTESIAN_POINT ( 'NONE',  ( -53.70442692472617807, -283.9190000381987034, -341.6604057112347732 ) ) ;
#20198=CARTESIAN_POINT ( 'NONE',  ( -41.16900876815732602, -273.0639740661492283, -193.6397803870029577 ) ) ;
#20199=CARTESIAN_POINT ( 'NONE',  ( -66.98382599163394957, -292.3251023065710115, -199.4057999223121271 ) ) ;
#20200=CARTESIAN_POINT ( 'NONE',  ( -30.96383551090100639, -284.2714936815391980, -194.8521535206214139 ) ) ;
#20201=CARTESIAN_POINT ( 'NONE',  ( -82.83673185939223060, -289.9889221217006252, -332.4573850137394970 ) ) ;
#20203=CARTESIAN_POINT ( 'NONE',  ( 3.629980534029428441, -288.8176293778209924, -330.8655263877317907 ) ) ;
#20207=CARTESIAN_POINT ( 'NONE',  ( -55.21708144420773579, -169.6647128743276198, -360.6205609466671262 ) ) ;
#20208=CARTESIAN_POINT ( 'NONE',  ( -41.51171161027219370, -284.6237506083643893, -346.6056163753486885 ) ) ;
#20209=CARTESIAN_POINT ( 'NONE',  ( 39.58706461736021254, -291.0523547857346784, -270.3937649182068981 ) ) ;
#20211=CARTESIAN_POINT ( 'NONE',  ( 33.41553229368502542, -280.2196921497937296, -251.1391125658965962 ) ) ;
#20212=CARTESIAN_POINT ( 'NONE',  ( 21.71167546289456141, -275.8835959873263732, -319.7417125813740881 ) ) ;
#20213=CARTESIAN_POINT ( 'NONE',  ( -73.71128243261479440, -279.5362303201901568, -335.7767905355797780 ) ) ;
#20214=CARTESIAN_POINT ( 'NONE',  ( -20.14603930832873502, -109.6676116220293835, -360.2926962469870773 ) ) ;
#20215=CARTESIAN_POINT ( 'NONE',  ( 39.12091579616689074, -280.1217208419323583, -269.9516809897648955 ) ) ;
#20216=CARTESIAN_POINT ( 'NONE',  ( -55.12427778965803782, -283.8425770811846292, -197.8119445251706168 ) ) ;
#20218=CARTESIAN_POINT ( 'NONE',  ( -101.4733360123586294, -298.8535885687790028, -229.6044339707148652 ) ) ;
#20219=CARTESIAN_POINT ( 'NONE',  ( 35.48627625942331321, -294.1214413835087953, -276.1984373020115413 ) ) ;
#20221=CARTESIAN_POINT ( 'NONE',  ( -95.49440411143764607, -289.8654624382443785, -225.4221983369952511 ) ) ;
#20222=CARTESIAN_POINT ( 'NONE',  ( 38.11712176391364437, -276.0181213643333535, -255.5530463461401780 ) ) ;
#20223=CARTESIAN_POINT ( 'NONE',  ( -67.05750530498295348, -273.6514624167348870, -203.6693107640952860 ) ) ;
#20230=CARTESIAN_POINT ( 'NONE',  ( -21.30727050855444915, -283.9214463001050603, -341.9474228160043481 ) ) ;
#20231=CARTESIAN_POINT ( 'NONE',  ( -96.04903109183956644, -280.9691240146350424, -222.0975020886282891 ) ) ;
#20232=CARTESIAN_POINT ( 'NONE',  ( -110.1079542799334661, -283.4963208918729833, -279.0744888805806454 ) ) ;
#20233=CARTESIAN_POINT ( 'NONE',  ( -39.76489218590018027, -281.8818463398827134, -196.1527423568188340 ) ) ;
#20234=CARTESIAN_POINT ( 'NONE',  ( 22.85829715218401503, -273.4440892567648689, -227.8343478696969555 ) ) ;
#20237=CARTESIAN_POINT ( 'NONE',  ( -45.62203281981695113, -277.9572555538766210, -346.8051306091561514 ) ) ;
#20241=CARTESIAN_POINT ( 'NONE',  ( -92.21611822576460327, -285.8115205227973661, -322.0250182851863769 ) ) ;
#20242=CARTESIAN_POINT ( 'NONE',  ( 24.55843368802369397, -293.2880014324734361, -309.4559428039779618 ) ) ;
#20243=CARTESIAN_POINT ( 'NONE',  ( -46.02251494838112222, -288.5079465466793636, -346.8206942528800596 ) ) ;
#20245=CARTESIAN_POINT ( 'NONE',  ( -70.41540975968770510, -283.8499598856743091, -204.1344171334308442 ) ) ;
#20246=B_SPLINE_CURVE_WITH_KNOTS ( 'NONE', 3,
 ( #72341, #57671, #14588, #36808, #86990, #22590, #50555, #15036, #363, #8389, #87903, #15973, #43896, #7460, #80354, #15495, #44366, #37268, #16428, #29249, #73729, #81282, #65728, #73277 ),
 .UNSPECIFIED., .F., .F.,
 ( 4, 2, 2, 2, 2, 2, 2, 2, 2, 2, 2, 4 ),
 ( 5.000000000000000311E-10, 0.06250000043739493971, 0.1250000003747898936, 0.2500000002495797458, 0.3750000001243696812, 0.4999999999991595057, 0.6249999998739494966, 0.7499999997487395431, 0.8124999996861346219, 0.8749999996235297006, 0.9374999995609246684, 0.9999999994983197471 ),
 .UNSPECIFIED. ) ;
#20247=CARTESIAN_POINT ( 'NONE',  ( -101.4961819897355326, -283.6174466731628172, -234.2070815833755830 ) ) ;
#20248=CARTESIAN_POINT ( 'NONE',  ( 14.78133465449043804, -286.5452018655301458, -322.9078900774871386 ) ) ;
#20249=CARTESIAN_POINT ( 'NONE',  ( -29.38644591958286867, -284.1543610972602210, -343.3765760133306912 ) ) ;
#20250=CARTESIAN_POINT ( 'NONE',  ( -4.884051664691080319, -274.6246261236256032, -337.9881186185056663 ) ) ;
#20251=CARTESIAN_POINT ( 'NONE',  ( 9.336930237074478001, -285.0815183135947564, -210.1320064114818820 ) ) ;
#20252=CARTESIAN_POINT ( 'NONE',  ( -36.24728794247184283, -300.0660086204491108, -195.3607361450893904 ) ) ;
#20253=CARTESIAN_POINT ( 'NONE',  ( -100.9530954106502918, -283.0891964050535421, -230.3159083355264158 ) ) ;
#20254=CARTESIAN_POINT ( 'NONE',  ( 21.51093134818863462, -281.8839828914335612, -226.7535934818088492 ) ) ;
#20255=CARTESIAN_POINT ( 'NONE',  ( 24.03308083390703231, -288.9637462017158214, -226.9434909888439904 ) ) ;
#20258=CARTESIAN_POINT ( 'NONE',  ( 3.470481103912061105, -296.4285759718682698, -334.0126682316591769 ) ) ;
#20259=CARTESIAN_POINT ( 'NONE',  ( -69.35447072460878815, -277.6307593900839947, -202.5364678026601268 ) ) ;
#20260=CARTESIAN_POINT ( 'NONE',  ( -98.90590571253842711, -289.1361088475414931, -316.3612160950274870 ) ) ;
#20261=CARTESIAN_POINT ( 'NONE',  ( -42.46538574669811794, -293.5177172726479284, -343.9830458395301775 ) ) ;
#20262=CARTESIAN_POINT ( 'NONE',  ( -1.712431984400921925, -279.2196941532208712, -206.0820488370908663 ) ) ;
#20263=CARTESIAN_POINT ( 'NONE',  ( -101.9557794382960054, -271.1299254082481411, -233.2935517564702081 ) ) ;
#20264=CARTESIAN_POINT ( 'NONE',  ( 6.960275742959275647, -293.9849750373294341, -211.7217249899602223 ) ) ;
#20265=CARTESIAN_POINT ( 'NONE',  ( -106.6379572354042153, -292.6233781216987495, -303.7686719486574134 ) ) ;
#20266=CARTESIAN_POINT ( 'NONE',  ( -67.88201864047690037, -296.1385260511578394, -200.3763282158968195 ) ) ;
#20267=CARTESIAN_POINT ( 'NONE',  ( 10.65080245116904756, -289.9764879404780800, -326.4925973908365222 ) ) ;
#20268=CARTESIAN_POINT ( 'NONE',  ( 37.07415536079328433, -291.5964136802967346, -254.9266840776168692 ) ) ;
#20270=CARTESIAN_POINT ( 'NONE',  ( -97.82291620412300404, -291.3977410869941309, -312.3045731723368021 ) ) ;
#20273=CARTESIAN_POINT ( 'NONE',  ( -60.31935898979723731, -292.5494406911891474, -200.8484088883652419 ) ) ;
#20275=CARTESIAN_POINT ( 'NONE',  ( -96.28323037451396260, -292.4187085568170232, -221.4132961256111685 ) ) ;
#20276=CARTESIAN_POINT ( 'NONE',  ( 37.17225381297330244, -279.4244343820826657, -258.7935268516100678 ) ) ;
#20277=CARTESIAN_POINT ( 'NONE',  ( 34.48317378039007508, -293.3791421944624744, -257.2460165173690712 ) ) ;
#20279=CARTESIAN_POINT ( 'NONE',  ( 12.99217136191258959, -280.7327945145713102, -212.0901871436865633 ) ) ;
#20280=CARTESIAN_POINT ( 'NONE',  ( -44.42149925063706917, -282.8059782237352806, -347.0670586021096824 ) ) ;
#20281=CARTESIAN_POINT ( 'NONE',  ( -83.70149274560351671, -287.6899482708562914, -329.1046116803624386 ) ) ;
#20282=CARTESIAN_POINT ( 'NONE',  ( 24.72811970642363377, -279.1355028338772968, -229.5473350224219473 ) ) ;
#20283=CARTESIAN_POINT ( 'NONE',  ( -99.32875553787344813, -283.1247177520060063, -228.0485062650273562 ) ) ;
#20285=CARTESIAN_POINT ( 'NONE',  ( 82.64890176555634582, -299.5541904835127980, -197.2582414438974183 ) ) ;
#20286=CARTESIAN_POINT ( 'NONE',  ( 34.67978178036037207, -279.7093679855465211, -244.9918006069261480 ) ) ;
#20288=CARTESIAN_POINT ( 'NONE',  ( 37.08020550198332188, -286.2398930654125024, -251.8443020218966808 ) ) ;
#20290=CARTESIAN_POINT ( 'NONE',  ( 32.55218939409179058, -294.8390308304022369, -246.5107223462067907 ) ) ;
#20291=CARTESIAN_POINT ( 'NONE',  ( -1.593354834055566771, -275.9418614453367695, -202.8284436475601922 ) ) ;
#20292=CARTESIAN_POINT ( 'NONE',  ( -96.90540231159040729, -277.6289693470893667, -312.6232530551527589 ) ) ;
#20293=CARTESIAN_POINT ( 'NONE',  ( -50.56844179464368239, -292.0543754327635497, -194.5056415199272521 ) ) ;
#20295=CARTESIAN_POINT ( 'NONE',  ( -98.63499239916552597, -282.0339844744931952, -314.6350897270917812 ) ) ;
#20297=CARTESIAN_POINT ( 'NONE',  ( -94.46693240886691001, -290.2567086306071928, -224.5141684049796709 ) ) ;
#20298=CARTESIAN_POINT ( 'NONE',  ( 27.82397031902284112, -292.0482342373182405, -307.5932637264006644 ) ) ;
#20301=CARTESIAN_POINT ( 'NONE',  ( -46.99639627251990248, -291.4338592455980006, -197.9402971924112933 ) ) ;
#20303=CARTESIAN_POINT ( 'NONE',  ( 34.45848030099739390, -279.0523547857346784, -270.3937649182068412 ) ) ;
#20304=CARTESIAN_POINT ( 'NONE',  ( -112.6554975795644822, -295.7980956059822688, -255.4392073734181281 ) ) ;
#20305=CARTESIAN_POINT ( 'NONE',  ( 24.09162375906011988, -280.2895622214054470, -314.7255741764288359 ) ) ;
#20306=CARTESIAN_POINT ( 'NONE',  ( -103.9791965945457264, -285.3752146068695765, -308.0548433018115588 ) ) ;
#20307=CARTESIAN_POINT ( 'NONE',  ( 34.01022539348792151, -287.5896662920519020, -285.8438323092013889 ) ) ;
#20308=CARTESIAN_POINT ( 'NONE',  ( 30.92757452963751064, -277.4420827589030409, -298.2461111548918780 ) ) ;
#20309=CARTESIAN_POINT ( 'NONE',  ( -100.1302118997567305, -294.0248495407202540, -310.8222952834495914 ) ) ;
#20310=CARTESIAN_POINT ( 'NONE',  ( -96.39954614722465465, -297.6939223965513861, -314.9930276175385870 ) ) ;
#20312=CARTESIAN_POINT ( 'NONE',  ( -36.47681003665820754, -275.8360326052328446, -343.7656315442935693 ) ) ;
#20315=CARTESIAN_POINT ( 'NONE',  ( -86.38511144096445094, -295.3786136268852829, -329.6948191837436752 ) ) ;
#20316=CARTESIAN_POINT ( 'NONE',  ( -18.07772876651895899, -290.7222077603793196, -342.3189431944356897 ) ) ;
#20318=CARTESIAN_POINT ( 'NONE',  ( 35.06248585260316020, -288.3375044101859430, -280.5283673644694318 ) ) ;
#20320=CARTESIAN_POINT ( 'NONE',  ( -2.486235461489079590, -279.5605503510006429, -201.9511362877977376 ) ) ;
#20321=CARTESIAN_POINT ( 'NONE',  ( -90.63544387885218612, -296.4348027574329763, -325.8698757792051310 ) ) ;
#20322=CARTESIAN_POINT ( 'NONE',  ( -111.3637151172544861, -288.4863830695507545, -286.5180601888026217 ) ) ;
#20323=CARTESIAN_POINT ( 'NONE',  ( -86.37858375892867002, -296.0450687006342037, -329.7002141604654071 ) ) ;
#20324=CARTESIAN_POINT ( 'NONE',  ( 34.34594285037675121, -294.0686313189999055, -284.2524581280596863 ) ) ;
#20325=DIRECTION ( 'NONE',  ( 0.000000000000000000, 0.000000000000000000, 1.000000000000000000 ) ) ;
#20328=CARTESIAN_POINT ( 'NONE',  ( 20.06419942736765805, -289.7587214170598031, -320.6527736922806753 ) ) ;
#20329=CARTESIAN_POINT ( 'NONE',  ( -111.2586520408596868, -280.6233781216988064, -305.9938812882205070 ) ) ;
#20330=CARTESIAN_POINT ( 'NONE',  ( 35.50984106711873522, -281.2130808109043869, -295.1429158361315785 ) ) ;
#20331=CARTESIAN_POINT ( 'NONE',  ( -0.3234896261980607091, -284.5588246227664513, -335.3971120059162558 ) ) ;
#20332=CARTESIAN_POINT ( 'NONE',  ( 32.18349895377764369, -285.7170984082435439, -238.5342635943641767 ) ) ;
#20333=CARTESIAN_POINT ( 'NONE',  ( -101.5583311862220199, -288.1238534277226790, -308.1129103196010419 ) ) ;
#20334=CARTESIAN_POINT ( 'NONE',  ( 2.866396278645666484, -278.3795293334136431, -334.6382620907512546 ) ) ;
#20335=EDGE_LOOP ( 'NONE', ( #35505, #7301 ) ) ;
#20336=CARTESIAN_POINT ( 'NONE',  ( -105.2677981959970737, -278.1945495722657142, -297.1014470992312795 ) ) ;
#20337=CARTESIAN_POINT ( 'NONE',  ( -3.094003029295910867, -279.8657562179079150, -205.7637337317640345 ) ) ;
#20338=CARTESIAN_POINT ( 'NONE',  ( -39.93865872692391150, -278.1636973334351524, -347.0210386357355787 ) ) ;
#20339=CARTESIAN_POINT ( 'NONE',  ( -99.09860598740684168, -277.9523840343671282, -225.0168795927410486 ) ) ;
#20340=CARTESIAN_POINT ( 'NONE',  ( -90.56249836145711640, -228.8796048916817938, -345.2664085948654247 ) ) ;
#20341=CARTESIAN_POINT ( 'NONE',  ( -46.86372918164011736, -274.8752907586663241, -194.1892650757026502 ) ) ;
#20343=CARTESIAN_POINT ( 'NONE',  ( -112.8610223001902426, -274.2148066845750236, -259.0666763222170630 ) ) ;
#20344=CARTESIAN_POINT ( 'NONE',  ( -4.829096099716510437, -282.9805209788416391, -202.7746430608542312 ) ) ;
#20345=CARTESIAN_POINT ( 'NONE',  ( 82.61707336526248469, -302.0539871969763226, -195.3101965168185075 ) ) ;
#20346=CARTESIAN_POINT ( 'NONE',  ( 22.23478622320949682, -288.0362202097271620, -227.5570762895314658 ) ) ;
#20347=CARTESIAN_POINT ( 'NONE',  ( -101.6726619282658248, -286.8488919766878098, -229.9197855791585141 ) ) ;
#20348=CARTESIAN_POINT ( 'NONE',  ( 33.12973779667621699, -286.6443033693179814, -250.9274074458705570 ) ) ;
#20349=CARTESIAN_POINT ( 'NONE',  ( -109.2476828459184759, -283.7114212697549647, -297.8785047394810022 ) ) ;
#20350=CARTESIAN_POINT ( 'NONE',  ( -46.53614222585672167, -278.3335305031370126, -197.0844433046759150 ) ) ;
#20351=CARTESIAN_POINT ( 'NONE',  ( 24.55101473945552115, -288.8522035838777811, -229.2783718491601519 ) ) ;
#20352=CARTESIAN_POINT ( 'NONE',  ( 18.50247568030931689, -279.3534957848438580, -222.2570678281635139 ) ) ;
#20353=CARTESIAN_POINT ( 'NONE',  ( -16.22324682259606732, -278.0886709919066107, -340.8080568013381253 ) ) ;
#20354=CARTESIAN_POINT ( 'NONE',  ( 16.58080453554351408, -276.7512609193424851, -319.6783793734903156 ) ) ;
#20355=CARTESIAN_POINT ( 'NONE',  ( -36.10870396393215742, -287.8319791788437669, -346.9671660871619565 ) ) ;
#20357=CARTESIAN_POINT ( 'NONE',  ( -61.17186062352296716, -284.1565611471980333, -343.4665442839381626 ) ) ;
#20358=CARTESIAN_POINT ( 'NONE',  ( -114.2653783477883280, -285.0850247193957898, -267.1232558986135928 ) ) ;
#20359=CARTESIAN_POINT ( 'NONE',  ( -8.492288266139274455, -282.8303592510270050, -337.4186413467698458 ) ) ;
#20363=CARTESIAN_POINT ( 'NONE',  ( -72.87571208577669779, -293.4469955150468650, -203.4312889108192053 ) ) ;
#20365=CARTESIAN_POINT ( 'NONE',  ( 10.82141655263135149, -291.3867604471241179, -210.8487498597131946 ) ) ;
#20367=CARTESIAN_POINT ( 'NONE',  ( -110.1182556951474822, -271.7185119488624423, -262.1769009944317759 ) ) ;
#20368=CARTESIAN_POINT ( 'NONE',  ( 22.20243145212455715, -293.5549947794885952, -319.0419260028627377 ) ) ;
#20369=CARTESIAN_POINT ( 'NONE',  ( -111.0002282934223388, -288.9854729676389979, -273.9233504028511561 ) ) ;
#20370=CARTESIAN_POINT ( 'NONE',  ( 9.507355118070325517, -290.9460687350726289, -212.9959346869703438 ) ) ;
#20371=CARTESIAN_POINT ( 'NONE',  ( -104.4043105776840576, -291.3563450861241790, -300.3150304319308930 ) ) ;
#20372=FACE_OUTER_BOUND ( 'NONE', #28244, .T. ) ;
#20373=CARTESIAN_POINT ( 'NONE',  ( -112.1162529703692314, -292.4695425237663926, -276.8077118694866385 ) ) ;
#20374=CARTESIAN_POINT ( 'NONE',  ( -111.9959173749538195, -288.4342144578347984, -279.5541570975560148 ) ) ;
#20375=CARTESIAN_POINT ( 'NONE',  ( -111.8132970794172962, -292.4328340594520341, -279.6665501502061488 ) ) ;
#20376=CARTESIAN_POINT ( 'NONE',  ( 17.94597146388631614, -287.8108963234392377, -222.3331904971062727 ) ) ;
#20377=CARTESIAN_POINT ( 'NONE',  ( 35.30401363080866162, -295.3041644976250382, -251.0079314282764926 ) ) ;
#20378=CARTESIAN_POINT ( 'NONE',  ( -114.1722217312759540, -271.7244848033647031, -270.3505797943694802 ) ) ;
#20380=CARTESIAN_POINT ( 'NONE',  ( 23.97355982315887246, -276.9388371821778492, -226.5344224396591812 ) ) ;
#20382=CARTESIAN_POINT ( 'NONE',  ( -93.57827538333187078, -295.0339150718002657, -322.7408510826488737 ) ) ;
#20383=CARTESIAN_POINT ( 'NONE',  ( -6.080875328583586814, -272.7086000561169499, -203.2736016389281701 ) ) ;
#20384=CARTESIAN_POINT ( 'NONE',  ( -95.59490970013662547, -275.9899914341070257, -316.7266888545676693 ) ) ;
#20385=CARTESIAN_POINT ( 'NONE',  ( -110.7393439293485642, -273.7929662064518084, -267.6377504097686710 ) ) ;
#20386=CARTESIAN_POINT ( 'NONE',  ( -108.1649983417875944, -297.7153431090846993, -290.3469967014856365 ) ) ;
#20388=CARTESIAN_POINT ( 'NONE',  ( -105.9608351776847144, -297.6943620034685978, -244.8374633001775464 ) ) ;
#20390=CARTESIAN_POINT ( 'NONE',  ( -4.189732732382841718, -284.5071157111722187, -202.6759742074747521 ) ) ;
#20391=CARTESIAN_POINT ( 'NONE',  ( -40.51797094619345785, -298.0111363078657405, -197.4177026184339070 ) ) ;
#20392=CARTESIAN_POINT ( 'NONE',  ( -40.81647239334181165, -286.0097118476170408, -193.3873677658204144 ) ) ;
#20393=CARTESIAN_POINT ( 'NONE',  ( -73.16779326350092560, -289.1805869427522566, -338.5098221935239167 ) ) ;
#20394=CARTESIAN_POINT ( 'NONE',  ( -77.35098809753694127, -299.4982394415907834, -206.5045311814060085 ) ) ;
#20395=CARTESIAN_POINT ( 'NONE',  ( -28.70916093807228364, -292.9424050465045752, -344.7471701519687599 ) ) ;
#20396=CARTESIAN_POINT ( 'NONE',  ( 12.89433644350913610, -279.9300911685031110, -212.2190553290860464 ) ) ;
#20397=CARTESIAN_POINT ( 'NONE',  ( -37.37352853689063181, -292.5523547857347353, -345.3611179825600175 ) ) ;
#20399=CARTESIAN_POINT ( 'NONE',  ( 24.56506794068272725, -286.8893215445875171, -309.7905812284823810 ) ) ;
#20402=CARTESIAN_POINT ( 'NONE',  ( -99.78969702237375827, -287.9905435754104701, -311.9206185007499812 ) ) ;
#20403=CARTESIAN_POINT ( 'NONE',  ( -107.8656598809634630, -274.3547632669784662, -248.8067601240361739 ) ) ;
#20404=CARTESIAN_POINT ( 'NONE',  ( -59.15145743101420095, -281.2005355267744449, -197.1290158828732046 ) ) ;
#20405=CARTESIAN_POINT ( 'NONE',  ( -111.5878040651456757, -294.4038743814309100, -283.5376433228851170 ) ) ;
#20406=CARTESIAN_POINT ( 'NONE',  ( 28.15106865862283669, -281.9904623679659039, -302.7201711499558314 ) ) ;
#20407=CARTESIAN_POINT ( 'NONE',  ( -97.34768214340299153, -297.3654946523606100, -222.1088421096634704 ) ) ;
#20408=CARTESIAN_POINT ( 'NONE',  ( -67.11706186295245402, -299.1747116739355192, -202.9371024031307797 ) ) ;
#20410=CARTESIAN_POINT ( 'NONE',  ( 31.33118711821918012, -283.1575354286335369, -240.2109073186401247 ) ) ;
#20411=CARTESIAN_POINT ( 'NONE',  ( -92.01258371637722178, -296.3054952123812882, -221.6322462927990955 ) ) ;
#20414=CARTESIAN_POINT ( 'NONE',  ( -29.24166137129510190, -284.9290526642578811, -344.6167773334036042 ) ) ;
#20416=CARTESIAN_POINT ( 'NONE',  ( -69.91165696735023971, -286.9809262143061801, -337.9199732462171255 ) ) ;
#20417=CARTESIAN_POINT ( 'NONE',  ( 39.21874136230186991, -274.8311757613735153, -276.8923980205372573 ) ) ;
#20418=CARTESIAN_POINT ( 'NONE',  ( 10.93239676687030837, -292.5752655871932575, -215.5340840883249314 ) ) ;
#20419=CARTESIAN_POINT ( 'NONE',  ( 24.72474253690069190, -283.6178104478464093, -310.1848575823437386 ) ) ;
#20420=CARTESIAN_POINT ( 'NONE',  ( 32.81603944175314780, -276.8497865366781525, -247.2985686333061039 ) ) ;
#20421=CARTESIAN_POINT ( 'NONE',  ( -61.03161698088980813, -284.7789006027329037, -343.0620464176307109 ) ) ;
#20422=CARTESIAN_POINT ( 'NONE',  ( -3.451609935358393333, -281.3892701338144775, -335.4796701952996614 ) ) ;
#20423=CARTESIAN_POINT ( 'NONE',  ( -88.92415308158687992, -281.3280777168766349, -215.8443851696565332 ) ) ;
#20424=CARTESIAN_POINT ( 'NONE',  ( -71.40471085081489377, -273.7813799926016145, -201.3052615688016544 ) ) ;
#20425=CARTESIAN_POINT ( 'NONE',  ( 29.09487630824069626, -275.8921433325166959, -309.2864479864536520 ) ) ;
#20426=CARTESIAN_POINT ( 'NONE',  ( 4.648432004541546370, -296.4005354107971471, -331.8277186633598603 ) ) ;
#20428=DIRECTION ( 'NONE',  ( -1.000000000000000000, -0.000000000000000000, -0.000000000000000000 ) ) ;
#20430=CARTESIAN_POINT ( 'NONE',  ( -104.8677544210669907, -294.2407672179093652, -304.8357088850556238 ) ) ;
#20431=CARTESIAN_POINT ( 'NONE',  ( 24.03267669443869892, -275.6092042692771429, -310.0924314130461426 ) ) ;
#20433=CARTESIAN_POINT ( 'NONE',  ( -3.518533633770426050, -296.1340106258576839, -338.7766237963248273 ) ) ;
#20434=CARTESIAN_POINT ( 'NONE',  ( 21.07485016374559095, -295.4286133554568323, -319.9142750130876607 ) ) ;
#20435=CARTESIAN_POINT ( 'NONE',  ( -109.8920098641454075, -292.7890840106984456, -251.9655124535315451 ) ) ;
#20436=CARTESIAN_POINT ( 'NONE',  ( -79.68995846552437001, -275.6253767907149381, -332.1223138632049086 ) ) ;
#20437=CARTESIAN_POINT ( 'NONE',  ( -95.93925932665489142, -281.1072399395815751, -224.4315488720263829 ) ) ;
#20438=CARTESIAN_POINT ( 'NONE',  ( -64.10919113912578382, -293.4837654725556035, -339.8766338976153634 ) ) ;
#20439=CARTESIAN_POINT ( 'NONE',  ( 35.40695193088384940, -283.1422870585941496, -249.1500865670410860 ) ) ;
#20441=CARTESIAN_POINT ( 'NONE',  ( -42.68298839893505914, -284.9035396823200017, -197.2341673077121413 ) ) ;
#20442=CARTESIAN_POINT ( 'NONE',  ( 191.3483536179935811, 269.5978400234172909, -139.1112103393494408 ) ) ;
#20444=CARTESIAN_POINT ( 'NONE',  ( -109.0010619064832156, -284.0337586821974014, -284.3976188413744239 ) ) ;
#20446=CARTESIAN_POINT ( 'NONE',  ( -0.5117588490551993052, -283.6541554314484870, -337.6444748426573028 ) ) ;
#20447=CARTESIAN_POINT ( 'NONE',  ( -106.3148956329049071, -283.7769125809925299, -237.0338465774220253 ) ) ;
#20448=CARTESIAN_POINT ( 'NONE',  ( -111.5967773064131876, -279.2483762994376661, -289.8807546587031538 ) ) ;
#20450=CARTESIAN_POINT ( 'NONE',  ( -112.3802523404528984, -279.8965311945877943, -284.2864536832291833 ) ) ;
#20451=CARTESIAN_POINT ( 'NONE',  ( 24.50481641118622278, -281.5954315467186575, -224.6629650787219532 ) ) ;
#20452=CARTESIAN_POINT ( 'NONE',  ( -6.941161984400256557, -271.9809262143061233, -207.3071070584150277 ) ) ;
#20453=CARTESIAN_POINT ( 'NONE',  ( 140.1412609228563042, 179.8917986951376236, -241.4356369855332787 ) ) ;
#20455=CARTESIAN_POINT ( 'NONE',  ( 24.55475842122751828, -276.9814485145686831, -228.2803643704477281 ) ) ;
#20456=CARTESIAN_POINT ( 'NONE',  ( -84.51206451544574350, -219.2010842044853689, -352.3091733033897981 ) ) ;
#20457=CARTESIAN_POINT ( 'NONE',  ( -41.10955073043210461, -278.0245956044685158, -195.8114693833978492 ) ) ;
#20458=CARTESIAN_POINT ( 'NONE',  ( 35.31145055632104857, -295.0290512471046327, -248.1014299877745941 ) ) ;
#20459=CARTESIAN_POINT ( 'NONE',  ( 33.74883734666483548, -292.6757340138491941, -253.2774021417273502 ) ) ;
#20460=CARTESIAN_POINT ( 'NONE',  ( -73.15079238616165469, -289.0215466378542146, -338.4731157773885002 ) ) ;
#20462=EDGE_CURVE ( 'NONE', #92893, #48357, #80777, .T. ) ;
#20463=CARTESIAN_POINT ( 'NONE',  ( 15.06130190458702067, -292.9046557263863519, -325.9716535823719141 ) ) ;
#20464=CARTESIAN_POINT ( 'NONE',  ( -14.29706308860500741, -284.7557386602671841, -200.1977050575218300 ) ) ;
#20465=CARTESIAN_POINT ( 'NONE',  ( -105.8520131514659681, -292.7912150865183776, -241.6404922226025178 ) ) ;
#20467=CARTESIAN_POINT ( 'NONE',  ( -110.5858853170589100, -285.7881341990832880, -276.4053559942871630 ) ) ;
#20469=CARTESIAN_POINT ( 'NONE',  ( -73.33403450289934256, -292.5279801310514358, -202.5423389306555180 ) ) ;
#20470=CARTESIAN_POINT ( 'NONE',  ( -16.10863393030117052, -283.2624068247573064, -340.2692386936687399 ) ) ;
#20471=CARTESIAN_POINT ( 'NONE',  ( 10.93610531442968892, -293.1964200974447294, -329.9043511323453686 ) ) ;
#20472=CARTESIAN_POINT ( 'NONE',  ( 31.54719535292074895, -288.7946355083011554, -304.5175835615713140 ) ) ;
#20473=CARTESIAN_POINT ( 'NONE',  ( -57.26890966671346206, -289.7948203679932249, -344.7292534169084206 ) ) ;
#20474=CARTESIAN_POINT ( 'NONE',  ( 20.35877036529091555, -288.3488345981965040, -315.0988680951542733 ) ) ;
#20477=CARTESIAN_POINT ( 'NONE',  ( -112.5515424773979731, -298.5289093366816928, -261.2076982133957586 ) ) ;
#20478=CARTESIAN_POINT ( 'NONE',  ( -59.98604504535602899, -296.4496552780331626, -197.2270128695543292 ) ) ;
#20479=CARTESIAN_POINT ( 'NONE',  ( -38.34507198342080869, -279.0980197211071641, -197.1202562168407724 ) ) ;
#20480=CARTESIAN_POINT ( 'NONE',  ( -24.16397506914693238, -273.7236238496915917, -194.5054476279020719 ) ) ;
#20482=CARTESIAN_POINT ( 'NONE',  ( -20.71034507222360332, -293.3147647427265952, -342.2058151733558020 ) ) ;
#20483=CARTESIAN_POINT ( 'NONE',  ( 34.57644041368872934, -277.5404733683647578, -287.9004279230227326 ) ) ;
#20484=CARTESIAN_POINT ( 'NONE',  ( -66.27305071856305574, -271.8088978262707087, -201.9956118050231453 ) ) ;
#20485=CARTESIAN_POINT ( 'NONE',  ( -35.62603008020256823, -296.2352632241772312, -343.7507013140864274 ) ) ;
#20486=CARTESIAN_POINT ( 'NONE',  ( -47.82369977251103421, -296.2681204860084563, -342.9684803419327181 ) ) ;
#20488=CARTESIAN_POINT ( 'NONE',  ( -81.39244645041365800, -297.2399530912869068, -332.6024950123676831 ) ) ;
#20489=CARTESIAN_POINT ( 'NONE',  ( -99.22646076874328003, -295.1292966932009563, -227.6734785380151607 ) ) ;
#20490=CARTESIAN_POINT ( 'NONE',  ( -20.05609399799226722, -292.9314918050943675, -199.2799061855964453 ) ) ;
#20491=CARTESIAN_POINT ( 'NONE',  ( -113.7033333701804878, -273.4621055185214686, -261.8136160753545028 ) ) ;
#20492=CARTESIAN_POINT ( 'NONE',  ( -90.22726264439558008, -289.8604473470688845, -219.1899132447925354 ) ) ;
#20493=CARTESIAN_POINT ( 'NONE',  ( -55.32532138856537784, -274.3191160726446469, -195.5539240142365145 ) ) ;
#20494=CARTESIAN_POINT ( 'NONE',  ( -101.2351153521751570, -297.3684484705749469, -235.0097534021477372 ) ) ;
#20495=CARTESIAN_POINT ( 'NONE',  ( 16.03975319350223216, -282.7838889098434834, -217.1012560017240105 ) ) ;
#20496=CARTESIAN_POINT ( 'NONE',  ( -3.858216683970966177, -279.1694462342545648, -201.5560330292473736 ) ) ;
#20497=CARTESIAN_POINT ( 'NONE',  ( -66.54523214032158762, -282.7733014816466834, -341.5122418298900584 ) ) ;
#20498=CARTESIAN_POINT ( 'NONE',  ( 21.64709106172834652, -275.5655154088543100, -319.6930072728634400 ) ) ;
#20499=CARTESIAN_POINT ( 'NONE',  ( 36.90270245428426676, -279.7346075005963257, -253.1511964099847773 ) ) ;
#20500=CARTESIAN_POINT ( 'NONE',  ( 21.08182723941909131, -280.2018833302793723, -317.6753896169302038 ) ) ;
#20501=CARTESIAN_POINT ( 'NONE',  ( -67.28073941702785987, -272.2264205976156859, -203.1235940001424183 ) ) ;
#20502=CARTESIAN_POINT ( 'NONE',  ( -35.01683794608413081, -279.0231413477883393, -345.3376455229458202 ) ) ;
#20503=CARTESIAN_POINT ( 'NONE',  ( 121.3395553409046670, -299.5541904835127980, -195.3611179825600175 ) ) ;
#20505=CARTESIAN_POINT ( 'NONE',  ( -3.942567235151725580, -296.7046938696523171, -194.3842891811289917 ) ) ;
#20506=CARTESIAN_POINT ( 'NONE',  ( -41.92811500392247837, -290.0147222715382895, -195.1456169040285431 ) ) ;
#20507=CARTESIAN_POINT ( 'NONE',  ( -88.64948411077057244, -291.3553147882960843, -212.9458647584758637 ) ) ;
#20509=CARTESIAN_POINT ( 'NONE',  ( 36.91245703652465693, -277.4016548826752455, -258.6014898098471804 ) ) ;
#20510=CARTESIAN_POINT ( 'NONE',  ( 32.03429725566758890, -273.1786910845457896, -241.7295174292877107 ) ) ;
#20512=CARTESIAN_POINT ( 'NONE',  ( 36.73867465573334101, -283.6619425252267206, -285.2410465099249564 ) ) ;
#20514=CARTESIAN_POINT ( 'NONE',  ( -109.0741376417059172, -282.8362388024168013, -248.2923273916712219 ) ) ;
#20517=CARTESIAN_POINT ( 'NONE',  ( 4.027608214087640803, -293.2758089049786463, -330.9887588017700182 ) ) ;
#20518=CARTESIAN_POINT ( 'NONE',  ( -9.000254227003669172, -284.5663571159282128, -201.7352234822287755 ) ) ;
#20520=CARTESIAN_POINT ( 'NONE',  ( -17.72116012565841814, -292.7989158357086126, -342.7492044050287632 ) ) ;
#20521=CARTESIAN_POINT ( 'NONE',  ( -91.95118824806618818, -282.2943464781878902, -323.6575677650159832 ) ) ;
#20522=CARTESIAN_POINT ( 'NONE',  ( -95.43306958051316258, -280.7872660989660858, -224.8233755152020876 ) ) ;
#20523=CARTESIAN_POINT ( 'NONE',  ( -112.6110239454851012, -285.9395592664937453, -255.8532544176854628 ) ) ;
#20524=CARTESIAN_POINT ( 'NONE',  ( 28.42095924687072639, -279.2903717269009007, -232.2921457894609603 ) ) ;
#20525=CARTESIAN_POINT ( 'NONE',  ( -8.254947446710065861, -286.4439793904407452, -203.4062016697698425 ) ) ;
#20526=CARTESIAN_POINT ( 'NONE',  ( -109.3375112250729728, -279.7781157698582888, -285.5919453840065216 ) ) ;
#20527=CARTESIAN_POINT ( 'NONE',  ( -98.13347169816687199, -279.9201761581308574, -229.5653423659223336 ) ) ;
#20528=CARTESIAN_POINT ( 'NONE',  ( -90.75528151023307544, -287.2790405708038861, -217.2066626127095219 ) ) ;
#20530=CARTESIAN_POINT ( 'NONE',  ( -35.82601815709919890, -297.9039588445401705, -193.3611594079439442 ) ) ;
#20531=CARTESIAN_POINT ( 'NONE',  ( -39.99162214153800221, -291.0653794007516808, -345.0095633290131900 ) ) ;
#20533=CARTESIAN_POINT ( 'NONE',  ( -106.6662871844225293, -275.4805209788417528, -237.0123917617630980 ) ) ;
#20535=CARTESIAN_POINT ( 'NONE',  ( -36.92372284428714124, -272.0572502180299352, -195.1828672871213541 ) ) ;
#20536=CARTESIAN_POINT ( 'NONE',  ( 37.54287019753216015, -291.7738682656586775, -256.2635457052647894 ) ) ;
#20537=CARTESIAN_POINT ( 'NONE',  ( -35.13913671767085845, -297.5881088752313417, -197.2997692740603952 ) ) ;
#20538=CARTESIAN_POINT ( 'NONE',  ( -87.18420506855721896, -291.2815427122679353, -324.7113769294397230 ) ) ;
#20539=CARTESIAN_POINT ( 'NONE',  ( 35.22863737886870439, -283.5023556844174664, -284.9687244640829817 ) ) ;
#20541=CARTESIAN_POINT ( 'NONE',  ( -96.00209079540667290, -291.2018441956485617, -319.4961638596646480 ) ) ;
#20542=CARTESIAN_POINT ( 'NONE',  ( -112.3091949344336484, -286.5806676303881773, -268.1530943802150091 ) ) ;
#20543=CARTESIAN_POINT ( 'NONE',  ( -35.33815598716348916, -280.2432961900918826, -193.3740517007247206 ) ) ;
#20544=CARTESIAN_POINT ( 'NONE',  ( -47.46333827471196543, -293.2596920061812966, -345.2401313140499610 ) ) ;
#20545=CARTESIAN_POINT ( 'NONE',  ( 32.39148862436221066, -281.8050054480718245, -303.1407087741107489 ) ) ;
#20546=CARTESIAN_POINT ( 'NONE',  ( 36.81959874666089405, -277.3565715043815203, -266.0439140182618303 ) ) ;
#20547=CARTESIAN_POINT ( 'NONE',  ( 30.89617123739170168, -277.8376638359844719, -254.7536222014695397 ) ) ;
#20548=CARTESIAN_POINT ( 'NONE',  ( 38.60947445830576896, -273.8383533252995790, -274.0178505739139609 ) ) ;
#20550=CARTESIAN_POINT ( 'NONE',  ( 17.11286042825096132, -280.3635147099731171, -221.6508595519935056 ) ) ;
#20551=CARTESIAN_POINT ( 'NONE',  ( -34.29146492694944470, -278.2196694269658224, -346.9032944910129004 ) ) ;
#20552=CARTESIAN_POINT ( 'NONE',  ( -5.106770209196980659, -275.8007882320975455, -204.3006068977298071 ) ) ;
#20553=CARTESIAN_POINT ( 'NONE',  ( -114.1054157559419195, -283.6157953064064827, -269.9710214781242144 ) ) ;
#20554=CARTESIAN_POINT ( 'NONE',  ( -107.5393938696417564, -292.6195669391524916, -246.9035433754005737 ) ) ;
#20555=CARTESIAN_POINT ( 'NONE',  ( -57.92531130860410826, -275.3908608601349783, -196.9390011479957820 ) ) ;
#20556=CARTESIAN_POINT ( 'NONE',  ( -113.8485494440449202, -273.8671145182713076, -270.3778261331385124 ) ) ;
#20558=CARTESIAN_POINT ( 'NONE',  ( -110.8512665761547851, -298.7335213448432683, -256.2794686918437606 ) ) ;
#20559=CARTESIAN_POINT ( 'NONE',  ( -59.51506101398956616, -281.3396374703711444, -341.8884658692127800 ) ) ;
#20560=CARTESIAN_POINT ( 'NONE',  ( -72.15890625234015943, -291.2710885767406239, -201.6915418408783296 ) ) ;
#20561=CARTESIAN_POINT ( 'NONE',  ( 16.77332832658423456, -274.2971306752575060, -321.7752259495853764 ) ) ;
#20562=CARTESIAN_POINT ( 'NONE',  ( -20.65157451555334589, -290.4415928164342517, -344.7649358072233099 ) ) ;
#20563=CARTESIAN_POINT ( 'NONE',  ( -60.34296287108740131, -290.6672399465470562, -200.7006164639592498 ) ) ;
#20565=CARTESIAN_POINT ( 'NONE',  ( -112.0599370379590169, -289.3291897885905541, -254.3059781325443964 ) ) ;
#20566=CARTESIAN_POINT ( 'NONE',  ( -108.1279254967938925, -290.4560197681713021, -252.3827060009795105 ) ) ;
#20568=CARTESIAN_POINT ( 'NONE',  ( 35.55091329399895272, -288.3287971700274284, -246.3552834759147743 ) ) ;
#20569=CARTESIAN_POINT ( 'NONE',  ( -109.3061973778969360, -278.7212299547822454, -282.8123436188760707 ) ) ;
#20570=CARTESIAN_POINT ( 'NONE',  ( -69.41123858578896488, -294.3846748009860903, -340.0392384753142210 ) ) ;
#20571=CARTESIAN_POINT ( 'NONE',  ( -114.2526729939563239, -285.1723432283396278, -272.8542163725981027 ) ) ;
#20572=CARTESIAN_POINT ( 'NONE',  ( -113.8823868297742621, -284.7828308592328312, -278.5627989511127112 ) ) ;
#20573=CARTESIAN_POINT ( 'NONE',  ( -3.607841525799501792, -282.9273782984321315, -335.1371091619191134 ) ) ;
#20574=CARTESIAN_POINT ( 'NONE',  ( -48.09564758678637730, -154.9642027764678289, -365.2473460210824214 ) ) ;
#20575=CARTESIAN_POINT ( 'NONE',  ( -105.0018845002311565, -254.6799856396871462, -325.8108064456704938 ) ) ;
#20576=CARTESIAN_POINT ( 'NONE',  ( -48.36594557731149280, -154.7337953574015899, -361.4374211060301718 ) ) ;
#20577=CARTESIAN_POINT ( 'NONE',  ( -110.5027959604814072, -271.7853810092052527, -267.6210354056324263 ) ) ;
#20578=CARTESIAN_POINT ( 'NONE',  ( 9.693896526445993089, -273.6373114254649863, -214.0640462950258893 ) ) ;
#20579=CARTESIAN_POINT ( 'NONE',  ( 11.15465836344534800, -293.9090339482976333, -330.1594115452946880 ) ) ;
#20580=CARTESIAN_POINT ( 'NONE',  ( -61.85293824084561720, -183.3176616290708978, -359.0448971616088443 ) ) ;
#20582=CARTESIAN_POINT ( 'NONE',  ( -102.2914863981954028, -271.7693718857182716, -229.9281668713755380 ) ) ;
#20583=CARTESIAN_POINT ( 'NONE',  ( -80.46449502298644063, -299.3210897720525736, -209.9352126245723866 ) ) ;
#20584=EDGE_CURVE ( 'NONE', #71834, #31036, #54802, .T. ) ;
#20585=CARTESIAN_POINT ( 'NONE',  ( -69.16416843489774635, -292.7031567126353480, -204.3051734595368316 ) ) ;
#20587=CARTESIAN_POINT ( 'NONE',  ( -65.46699705325973184, -298.6346813656243739, -198.8774979795657885 ) ) ;
#20588=CARTESIAN_POINT ( 'NONE',  ( 35.71677250282696292, -288.0533248545674496, -271.0304596698283603 ) ) ;
#20589=CARTESIAN_POINT ( 'NONE',  ( -30.59492504527749901, -295.7717194548351927, -346.9028702906401804 ) ) ;
#20590=CARTESIAN_POINT ( 'NONE',  ( -8.405358854199741714, -295.1758240623362894, -341.7072127273230535 ) ) ;
#20591=CARTESIAN_POINT ( 'NONE',  ( 22.58672043617612601, -293.1375790046675434, -228.6547514383005932 ) ) ;
#20593=CARTESIAN_POINT ( 'NONE',  ( 20.72819778475617625, -276.8096241888264899, -222.0165096189973610 ) ) ;
#20595=CARTESIAN_POINT ( 'NONE',  ( -109.5462627524148900, -278.3976335827215962, -243.6361517084054356 ) ) ;
#20596=CARTESIAN_POINT ( 'NONE',  ( -14.00176467120770241, -275.3037913642411922, -200.9445791702334532 ) ) ;
#20597=CARTESIAN_POINT ( 'NONE',  ( 17.34453868686904698, -276.5795275588117761, -217.5277734039811719 ) ) ;
#20598=CARTESIAN_POINT ( 'NONE',  ( -112.5908924339967285, -276.5211947720129615, -274.3568478868846796 ) ) ;
#20599=CARTESIAN_POINT ( 'NONE',  ( -90.12520409805796362, -297.9330644373174550, -219.7140250709381348 ) ) ;
#20600=CARTESIAN_POINT ( 'NONE',  ( -106.5474714951690487, -294.7944984498337249, -295.5297720092256100 ) ) ;
#20602=CARTESIAN_POINT ( 'NONE',  ( -106.1233782964871750, -279.4896621579867997, -235.7662531688034733 ) ) ;
#20603=CARTESIAN_POINT ( 'NONE',  ( -8.736720786006902273, -276.8338497945538279, -337.5368163789413529 ) ) ;
#20604=CARTESIAN_POINT ( 'NONE',  ( -12.84565473796202362, -285.0488624312961292, -197.8818655564179210 ) ) ;
#20605=CARTESIAN_POINT ( 'NONE',  ( -79.61551375678384090, -299.4829905163437616, -208.1458641003685273 ) ) ;
#20607=CARTESIAN_POINT ( 'NONE',  ( -0.9199129578981691813, -287.7528504982832942, -333.8706304382895382 ) ) ;
#20608=CARTESIAN_POINT ( 'NONE',  ( -16.61678434090731571, -278.5634683795046271, -199.3086593551412307 ) ) ;
#20609=CARTESIAN_POINT ( 'NONE',  ( -110.2026008664295915, -277.2666439599022397, -259.6803181408615160 ) ) ;
#20610=CARTESIAN_POINT ( 'NONE',  ( -40.31589792167037700, -281.1696790036205584, -344.7416822955788120 ) ) ;
#20611=CARTESIAN_POINT ( 'NONE',  ( 37.47492556833609001, -289.4762135491798745, -264.4340648264293350 ) ) ;
#20612=CARTESIAN_POINT ( 'NONE',  ( -4.876711406066927879, -277.8199528496396056, -336.2017895178984759 ) ) ;
#20614=CARTESIAN_POINT ( 'NONE',  ( -104.0962041061745538, -276.3160045221297310, -306.6627737323630640 ) ) ;
#20615=CARTESIAN_POINT ( 'NONE',  ( -36.74355774891985504, -274.7112778488695994, -197.2491995169925474 ) ) ;
#20616=CARTESIAN_POINT ( 'NONE',  ( 3.569741778591647208, -284.5038572337506366, -333.4804175768238110 ) ) ;
#20618=CARTESIAN_POINT ( 'NONE',  ( 13.65029814504605987, -290.2649952785097298, -326.1916170002156150 ) ) ;
#20619=CARTESIAN_POINT ( 'NONE',  ( -23.47894108206374852, -290.2290642114985530, -196.6013032327773544 ) ) ;
#20620=CARTESIAN_POINT ( 'NONE',  ( 82.15666016531748994, -298.9416642213269029, -197.2723373383452383 ) ) ;
#20621=CARTESIAN_POINT ( 'NONE',  ( 22.69329040579045298, -273.6490041103211297, -227.9477779744090071 ) ) ;
#20622=CARTESIAN_POINT ( 'NONE',  ( -1.828028687576657818, -290.6674034986428978, -205.1573821108576112 ) ) ;
#20623=CARTESIAN_POINT ( 'NONE',  ( 68.56402772857219929, 46.98157435473511612, -321.4867780223927980 ) ) ;
#20625=CARTESIAN_POINT ( 'NONE',  ( -109.2190586751007402, -288.7039528740641003, -296.1372691806154762 ) ) ;
#20626=CARTESIAN_POINT ( 'NONE',  ( -91.31276540261265495, -285.4362405398349551, -320.6956441906409623 ) ) ;
#20627=CARTESIAN_POINT ( 'NONE',  ( 35.40865071816693899, -286.0715831718487152, -292.3461931515810761 ) ) ;
#20628=CARTESIAN_POINT ( 'NONE',  ( -93.86307815798451770, -285.3140703446956650, -317.4855144701957101 ) ) ;
#20629=CARTESIAN_POINT ( 'NONE',  ( -108.5801924970181744, -285.1349949749995289, -287.0795220944924608 ) ) ;
#20630=CARTESIAN_POINT ( 'NONE',  ( -112.6072130482546214, -292.4850761205244680, -274.0366267838651879 ) ) ;
#20631=CARTESIAN_POINT ( 'NONE',  ( 37.30912635175043590, -273.7851145521747185, -282.3750768043902895 ) ) ;
#20632=CARTESIAN_POINT ( 'NONE',  ( 26.05188392677884224, -276.4631487834815289, -314.1225709385395248 ) ) ;
#20633=CARTESIAN_POINT ( 'NONE',  ( -112.3864280376646860, -288.5142079795967334, -279.6034059470242141 ) ) ;
#20634=CARTESIAN_POINT ( 'NONE',  ( -67.70860737833254461, -277.4397783517609355, -341.1202230083772520 ) ) ;
#20635=CARTESIAN_POINT ( 'NONE',  ( -61.52267975163120894, -297.3475836450063525, -341.0354864051587924 ) ) ;
#20638=CARTESIAN_POINT ( 'NONE',  ( -85.19548484829935830, -282.4143702902513837, -326.1397766668883378 ) ) ;
#20639=CARTESIAN_POINT ( 'NONE',  ( -50.56142015072196472, -277.8831487152559703, -196.5353795947974049 ) ) ;
#20641=CARTESIAN_POINT ( 'NONE',  ( 38.92947524948860405, -274.0783339532729883, -274.0301079433759810 ) ) ;
#20642=CARTESIAN_POINT ( 'NONE',  ( -37.81873970715011524, -276.4068319517576811, -343.4739650071252299 ) ) ;
#20643=CARTESIAN_POINT ( 'NONE',  ( -2.801818328652338597, -296.1069215368674463, -335.4587701603929304 ) ) ;
#20644=CARTESIAN_POINT ( 'NONE',  ( 39.31041463148132920, -280.5031009006950171, -272.7995215156219615 ) ) ;
#20645=CARTESIAN_POINT ( 'NONE',  ( -94.11737487915920042, -296.8404814350064953, -316.6402141705581812 ) ) ;
#20646=CARTESIAN_POINT ( 'NONE',  ( 0.3124782378701334573, -295.8766939259398328, -336.9754596470872343 ) ) ;
#20647=CARTESIAN_POINT ( 'NONE',  ( 94.41209358101258431, -299.5800556217366193, -197.3651080369727708 ) ) ;
#20648=CARTESIAN_POINT ( 'NONE',  ( -69.90847475729853500, -293.6234967485889342, -202.7865481686931162 ) ) ;
#20649=CARTESIAN_POINT ( 'NONE',  ( -114.1520200293542473, -284.7952553521871550, -264.2503526948493118 ) ) ;
#20650=CARTESIAN_POINT ( 'NONE',  ( -13.42950850562544929, -272.4989993467435738, -198.4687500235213804 ) ) ;
#20651=CARTESIAN_POINT ( 'NONE',  ( 16.30070993815878566, -286.6220970128609338, -215.1208080017152326 ) ) ;
#20652=CARTESIAN_POINT ( 'NONE',  ( -96.93989397299300492, -281.1496530507380385, -225.3965717038308014 ) ) ;
#20653=CARTESIAN_POINT ( 'NONE',  ( -67.63411484682815455, -284.7033705575130398, -203.6844499546599536 ) ) ;
#20654=CARTESIAN_POINT ( 'NONE',  ( -36.14498329869359594, -287.0370230935881182, -345.3643443442269927 ) ) ;
#20655=CARTESIAN_POINT ( 'NONE',  ( -65.60899210820664962, -198.9355752380678553, -358.8784014864789924 ) ) ;
#20656=CARTESIAN_POINT ( 'NONE',  ( 6.969220374530967099, -286.1813703017011790, -212.2064806298952249 ) ) ;
#20657=CARTESIAN_POINT ( 'NONE',  ( -53.32857801162950295, -290.9108321976858633, -195.2252330318355860 ) ) ;
#20658=CARTESIAN_POINT ( 'NONE',  ( -113.5778603670490128, -280.1723693397156580, -268.7714838195372522 ) ) ;
#20659=CARTESIAN_POINT ( 'NONE',  ( -112.3070299301571993, -279.6741693204269268, -285.7064214304120355 ) ) ;
#20660=CARTESIAN_POINT ( 'NONE',  ( 24.12929439058094871, -281.9312803662752458, -309.8281039256343092 ) ) ;
#20661=CARTESIAN_POINT ( 'NONE',  ( -29.81377501960339771, -276.1476309346280118, -195.7398677138005780 ) ) ;
#20662=CARTESIAN_POINT ( 'NONE',  ( -68.22617953468768803, -295.4467134199439329, -340.8958536224056388 ) ) ;
#20663=CARTESIAN_POINT ( 'NONE',  ( -5.104402729032415209, -286.6457822885271298, -337.6857305970476091 ) ) ;
#20664=CARTESIAN_POINT ( 'NONE',  ( -107.1679009692855402, -295.1756813818711862, -292.8532874764903795 ) ) ;
#20666=CARTESIAN_POINT ( 'NONE',  ( -56.66968670148714438, -285.2234287546890528, -342.2481344050952998 ) ) ;
#20667=CARTESIAN_POINT ( 'NONE',  ( -63.58055407155491423, -295.0703823581748679, -338.5587319541636475 ) ) ;
#20668=CARTESIAN_POINT ( 'NONE',  ( -8.639715598758026971, -293.4987615638497118, -199.2436897807114349 ) ) ;
#20669=CARTESIAN_POINT ( 'NONE',  ( -38.87891642067148723, -283.7233205021925073, -343.4593954369836979 ) ) ;
#20671=CARTESIAN_POINT ( 'NONE',  ( -32.68486343263671756, -273.1682157176454666, -193.7246816214905323 ) ) ;
#20672=CARTESIAN_POINT ( 'NONE',  ( 3.133547090913871624, -289.1754214415847173, -335.8075846623377174 ) ) ;
#20673=CARTESIAN_POINT ( 'NONE',  ( -35.94609271736964473, -281.1744479031477226, -346.1259737302938788 ) ) ;
#20674=CARTESIAN_POINT ( 'NONE',  ( -112.2976526568304649, -291.1047519415854481, -252.8297326358438966 ) ) ;
#20675=CARTESIAN_POINT ( 'NONE',  ( 23.52946783180308898, -288.4452092015594076, -310.7174236836295336 ) ) ;
#20677=CARTESIAN_POINT ( 'NONE',  ( 128.9467878515196162, -299.5541904835127980, -198.8526868767648352 ) ) ;
#20678=CARTESIAN_POINT ( 'NONE',  ( -38.83267329410574575, -140.1998172465924313, -360.9197421274957378 ) ) ;
#20679=CARTESIAN_POINT ( 'NONE',  ( -4.771743288812454686, -289.9809262143061801, -202.8022627189028810 ) ) ;
#20681=CARTESIAN_POINT ( 'NONE',  ( -102.4240027089262810, -277.9307569353740064, -236.5087154671401777 ) ) ;
#20682=CARTESIAN_POINT ( 'NONE',  ( 35.71123962399595086, -274.9113823402823300, -245.9234868334324062 ) ) ;
#20683=CARTESIAN_POINT ( 'NONE',  ( -111.4407549128927002, -280.6915240882544254, -259.5432454525962385 ) ) ;
#20684=CARTESIAN_POINT ( 'NONE',  ( -45.97742063028599802, -156.0892642442967713, -362.7395337765181011 ) ) ;
#20686=CARTESIAN_POINT ( 'NONE',  ( 8.209942395161199613, -279.2359934933105023, -208.9467070802182036 ) ) ;
#20687=CARTESIAN_POINT ( 'NONE',  ( -90.07370503217666169, -281.8214467921291089, -323.2653367409481575 ) ) ;
#20688=CARTESIAN_POINT ( 'NONE',  ( -92.93263769845842148, -297.5964752944574911, -322.1839592232947780 ) ) ;
#20689=CARTESIAN_POINT ( 'NONE',  ( 33.83679862977677288, -294.2623806580214705, -286.8968421600630450 ) ) ;
#20691=CARTESIAN_POINT ( 'NONE',  ( -109.7597976945589693, -289.4048864911461010, -257.5464503063615780 ) ) ;
#20692=CARTESIAN_POINT ( 'NONE',  ( 2.358265231522841177, -275.2209044652397552, -204.5035023488277943 ) ) ;
#20693=CARTESIAN_POINT ( 'NONE',  ( -102.0304462058307422, -273.0138301201752142, -236.4231523912723674 ) ) ;
#20698=CARTESIAN_POINT ( 'NONE',  ( -39.72499874009503174, -281.1012280292210903, -197.0781832256423058 ) ) ;
#20699=CARTESIAN_POINT ( 'NONE',  ( -66.98805117935783926, -281.4290139896001506, -200.3963562490588117 ) ) ;
#20700=CARTESIAN_POINT ( 'NONE',  ( -82.95059137580459208, -282.7523340880581486, -327.7257419291232168 ) ) ;
#20701=CARTESIAN_POINT ( 'NONE',  ( 34.64770173359642058, -283.1767846151940375, -252.1879640621988017 ) ) ;
#20702=CARTESIAN_POINT ( 'NONE',  ( -4.776966075357743868, -275.0951963103696016, -336.4829738990276837 ) ) ;
#20703=FACE_OUTER_BOUND ( 'NONE', #31970, .T. ) ;
#20705=CARTESIAN_POINT ( 'NONE',  ( -35.70467828869394111, -277.8349667625615780, -347.1952981290345406 ) ) ;
#20707=ORIENTED_EDGE ( 'NONE', *, *, #16197, .F. ) ;
#20709=CARTESIAN_POINT ( 'NONE',  ( -41.45361806466899424, -285.0834465771308146, -345.6552603841092264 ) ) ;
#20710=CARTESIAN_POINT ( 'NONE',  ( 23.48116052620613203, -292.1859238670654122, -229.7017851198063454 ) ) ;
#20711=CARTESIAN_POINT ( 'NONE',  ( -28.99649650406889734, -288.2977377251822872, -346.8584760208775037 ) ) ;
#20712=CARTESIAN_POINT ( 'NONE',  ( -10.35995967590083033, -284.6489722053108267, -201.4274510843903556 ) ) ;
#20713=CARTESIAN_POINT ( 'NONE',  ( -109.5032299632216137, -283.3156465319873973, -255.9358439664611922 ) ) ;
#20714=CARTESIAN_POINT ( 'NONE',  ( -5.374778843717738397, -286.8654976820677689, -337.1150688794369330 ) ) ;
#20715=CARTESIAN_POINT ( 'NONE',  ( -16.00248016678046525, -283.9750205940136993, -340.5876670606424454 ) ) ;
#20716=CARTESIAN_POINT ( 'NONE',  ( -30.00842227774316484, -272.1448144038657802, -195.7204877319498166 ) ) ;
#20717=CARTESIAN_POINT ( 'NONE',  ( -113.5259403506055662, -282.9928859177989580, -267.1278141250662088 ) ) ;
#20718=CARTESIAN_POINT ( 'NONE',  ( -92.20852106584543151, -297.8364558175825891, -321.5135038868004358 ) ) ;
#20719=CARTESIAN_POINT ( 'NONE',  ( -63.87561090928890906, -283.7068214045204400, -200.0196279862317397 ) ) ;
#20720=CARTESIAN_POINT ( 'NONE',  ( -110.3941962026603676, -279.5614070086731999, -265.1899222917380712 ) ) ;
#20721=CARTESIAN_POINT ( 'NONE',  ( 23.21089669944873535, -288.9462715007371116, -225.8256102786311317 ) ) ;
#20724=CARTESIAN_POINT ( 'NONE',  ( 30.93942987269103284, -295.8962521824159353, -302.8405713993465156 ) ) ;
#20725=CARTESIAN_POINT ( 'NONE',  ( -40.61794608402050244, -275.0931724838617924, -345.3023351529357114 ) ) ;
#20726=CARTESIAN_POINT ( 'NONE',  ( -86.40205771588632899, -290.5883884781811730, -211.1545715365120657 ) ) ;
#20727=CARTESIAN_POINT ( 'NONE',  ( 17.66337529269165074, -292.6484605857987162, -319.5826248361901776 ) ) ;
#20728=CARTESIAN_POINT ( 'NONE',  ( -34.27610397999585956, -278.7762859959636330, -196.9193022093285208 ) ) ;
#20729=CARTESIAN_POINT ( 'NONE',  ( -50.14403857545830334, -296.0266086211211700, -197.2381694088662698 ) ) ;
#20730=CARTESIAN_POINT ( 'NONE',  ( -3.423451136932255778, -293.8250127401769873, -205.1629902137349575 ) ) ;
#20731=CARTESIAN_POINT ( 'NONE',  ( 35.77081079830085031, -283.8376638359844719, -253.6410175316879361 ) ) ;
#20732=CARTESIAN_POINT ( 'NONE',  ( -70.41090225979451134, -296.1039986695323023, -201.5924068826096516 ) ) ;
#20733=CARTESIAN_POINT ( 'NONE',  ( -85.18837032191426317, -291.3255891978590171, -326.6169565860685111 ) ) ;
#20734=CARTESIAN_POINT ( 'NONE',  ( -67.90040479831368714, -289.8963981491785376, -200.7758306376524047 ) ) ;
#20735=CARTESIAN_POINT ( 'NONE',  ( -109.2904588517238267, -292.1796265437973830, -254.9095472839576928 ) ) ;
#20737=CARTESIAN_POINT ( 'NONE',  ( -66.63810330690455430, -292.4611100834927697, -203.3214096886038078 ) ) ;
#20739=CARTESIAN_POINT ( 'NONE',  ( -95.37021874277319000, -292.4361418703693403, -220.3340665504157414 ) ) ;
#20740=CARTESIAN_POINT ( 'NONE',  ( 29.60410717336755937, -280.0279259554579880, -304.9539739589831129 ) ) ;
#20741=CARTESIAN_POINT ( 'NONE',  ( -4.833079267209935637, -292.4925839043611973, -204.9852046106930175 ) ) ;
#20742=CARTESIAN_POINT ( 'NONE',  ( 36.17570850998654919, -281.2645293550647239, -247.4659082839496591 ) ) ;
#20743=CARTESIAN_POINT ( 'NONE',  ( 0.8541787609222049049, -282.2238465905517160, -337.2106116602250268 ) ) ;
#20744=CARTESIAN_POINT ( 'NONE',  ( 10.32058661838865987, -284.7097257661956178, -212.4533718015969725 ) ) ;
#20745=CARTESIAN_POINT ( 'NONE',  ( 18.51896090282600227, -280.3777764790950755, -319.2533671761889877 ) ) ;
#20746=CARTESIAN_POINT ( 'NONE',  ( -36.56000823155557811, -284.0618060800927651, -195.3524865577254275 ) ) ;
#20748=CARTESIAN_POINT ( 'NONE',  ( -19.89575639285349595, -278.7522021942000379, -196.0212611830721414 ) ) ;
#20749=CARTESIAN_POINT ( 'NONE',  ( -57.66074642615794232, -284.7162334006808351, -196.3558130224410547 ) ) ;
#20750=CARTESIAN_POINT ( 'NONE',  ( -24.57829108891397141, -275.0219112077140267, -198.2698641523999186 ) ) ;
#20752=CARTESIAN_POINT ( 'NONE',  ( 36.00436258126122624, -295.2648036968413976, -278.9839979288634595 ) ) ;
#20753=CARTESIAN_POINT ( 'NONE',  ( -31.32470331478227976, -275.5519792272103814, -194.1744386914177483 ) ) ;
#20754=CARTESIAN_POINT ( 'NONE',  ( -110.3014391925587887, -278.1793846025415178, -273.3551056796637795 ) ) ;
#20755=CARTESIAN_POINT ( 'NONE',  ( -84.26803050584193500, -291.5936904634081657, -209.2454148529283771 ) ) ;
#20756=CARTESIAN_POINT ( 'NONE',  ( 21.76448100599156277, -278.9896011899159589, -223.2685349867159914 ) ) ;
#20757=CARTESIAN_POINT ( 'NONE',  ( -72.17036813410757645, -291.4376627662732631, -201.6736429756137454 ) ) ;
#20758=CARTESIAN_POINT ( 'NONE',  ( -57.70891937894879931, -290.8414966902099081, -199.9618948131748368 ) ) ;
#20759=CARTESIAN_POINT ( 'NONE',  ( -4.137748087443496203, -292.6142979437767622, -337.6248627875890520 ) ) ;
#20762=CARTESIAN_POINT ( 'NONE',  ( 28.79689196603782975, -292.6394019826446993, -239.1985781341939514 ) ) ;
#20764=CARTESIAN_POINT ( 'NONE',  ( -109.1418805571601069, -276.0523547857346784, -270.3284710469131937 ) ) ;
#20765=CARTESIAN_POINT ( 'NONE',  ( -106.2966940996912939, -296.0454374831130053, -236.6264322918149219 ) ) ;
#20766=CARTESIAN_POINT ( 'NONE',  ( -94.95227913953195298, -285.1820416947531953, -320.7031427688282292 ) ) ;
#20767=CARTESIAN_POINT ( 'NONE',  ( 0.1704845652020387514, -286.3996527890865877, -207.6776213788750169 ) ) ;
#20768=CARTESIAN_POINT ( 'NONE',  ( 36.33569530298197492, -277.0522532264325264, -268.8284232869652328 ) ) ;
#20769=CARTESIAN_POINT ( 'NONE',  ( -98.54615216451782089, -293.9896120425282788, -313.0912227646948054 ) ) ;
#20770=CARTESIAN_POINT ( 'NONE',  ( -106.7640101030666528, -298.6515164449539839, -244.5515823946464593 ) ) ;
#20771=CARTESIAN_POINT ( 'NONE',  ( -13.67178574940730762, -275.5330076962840735, -339.8901880931460937 ) ) ;
#20774=CARTESIAN_POINT ( 'NONE',  ( -69.52294920914108900, -295.1309442718950322, -340.3048797477754874 ) ) ;
#20775=CARTESIAN_POINT ( 'NONE',  ( 20.65040558188598396, -290.1193487647574329, -317.0326283204814786 ) ) ;
#20776=CARTESIAN_POINT ( 'NONE',  ( 60.24221760881081167, -297.2734843241957492, -195.3943839220979442 ) ) ;
#20777=CARTESIAN_POINT ( 'NONE',  ( -15.81372404671005683, -289.4177381614483693, -340.2741573733025575 ) ) ;
#20780=CARTESIAN_POINT ( 'NONE',  ( -88.76491776713821480, -278.4094828741769447, -213.3657418541260142 ) ) ;
#20781=CARTESIAN_POINT ( 'NONE',  ( -100.6714333068340466, -297.7804423898321602, -226.7185096576982062 ) ) ;
#20782=CARTESIAN_POINT ( 'NONE',  ( -108.7101548051434889, -288.3637137330772475, -295.9500226618915235 ) ) ;
#20783=CARTESIAN_POINT ( 'NONE',  ( -68.21380337838547803, -295.7799407258559086, -340.8781906139090552 ) ) ;
#20784=CARTESIAN_POINT ( 'NONE',  ( 14.33424181413710130, -294.6345595904641641, -322.0237333995472682 ) ) ;
#20788=CARTESIAN_POINT ( 'NONE',  ( -37.48071883607661903, -290.5739415982342848, -346.6806149350667283 ) ) ;
#20789=CARTESIAN_POINT ( 'NONE',  ( 25.22466315766300227, -284.6948066931273047, -320.2154176792147382 ) ) ;
#20791=CARTESIAN_POINT ( 'NONE',  ( 37.09105149305234761, -281.1428124644008335, -289.6763522041675287 ) ) ;
#20792=CARTESIAN_POINT ( 'NONE',  ( -59.46645619217912326, -285.3393142992701428, -341.9035144645726518 ) ) ;
#20793=CARTESIAN_POINT ( 'NONE',  ( 37.97914149102219739, -285.9638418723594100, -257.4241356919386021 ) ) ;
#20794=CARTESIAN_POINT ( 'NONE',  ( -108.7702767015497045, -288.9044534800641486, -249.3570768277865000 ) ) ;
#20795=CARTESIAN_POINT ( 'NONE',  ( 37.69748899773254891, -277.2796082793372534, -259.9004499528941778 ) ) ;
#20797=CARTESIAN_POINT ( 'NONE',  ( -94.45303514320988825, -277.9098345345587404, -315.8486053523699297 ) ) ;
#20798=CARTESIAN_POINT ( 'NONE',  ( 34.66893093770704581, -280.7349615901142670, -257.7769341837247907 ) ) ;
#20799=CARTESIAN_POINT ( 'NONE',  ( 9.311370640959509615, -275.7561441169557952, -209.4925423733004664 ) ) ;
#20800=CARTESIAN_POINT ( 'NONE',  ( -72.31178479362132805, -278.3948331338272055, -202.1915589963417972 ) ) ;
#20801=CARTESIAN_POINT ( 'NONE',  ( 171.9668532218946950, 242.4161052218647683, -177.9424729848912534 ) ) ;
#20802=CARTESIAN_POINT ( 'NONE',  ( -15.85474592014891471, -275.2646036841996420, -196.6097434540513689 ) ) ;
#20804=CARTESIAN_POINT ( 'NONE',  ( -77.90515536138023833, -298.9437089510076362, -205.6060997081535504 ) ) ;
#20805=CARTESIAN_POINT ( 'NONE',  ( -20.25526795762937127, -288.7662352645560304, -195.3538533559490702 ) ) ;
#20807=CARTESIAN_POINT ( 'NONE',  ( 35.86041165532898134, -288.5686672958799477, -265.5527860586612974 ) ) ;
#20808=CARTESIAN_POINT ( 'NONE',  ( -5.222919879042626334, -288.2292120952364485, -201.4963376337424563 ) ) ;
#20810=CARTESIAN_POINT ( 'NONE',  ( -10.69466430851150207, -288.0439238285759984, -338.4876342318938782 ) ) ;
#20811=CARTESIAN_POINT ( 'NONE',  ( -113.7577895998465465, -284.1718320527639889, -261.4108010605994536 ) ) ;
#20812=CARTESIAN_POINT ( 'NONE',  ( 9.803081668116483627, -279.1133610424893732, -213.5158808613807935 ) ) ;
#20813=CARTESIAN_POINT ( 'NONE',  ( 3.100423554835791684, -288.4621026972658910, -208.1092094905771432 ) ) ;
#20814=CARTESIAN_POINT ( 'NONE',  ( 35.25339923136706943, -279.8663931735749770, -257.6859729172309130 ) ) ;
#20815=CARTESIAN_POINT ( 'NONE',  ( -93.97541681768129251, -279.2075490431035973, -317.2195489370879500 ) ) ;
#20816=CARTESIAN_POINT ( 'NONE',  ( 2.958663204777464362, -275.1013428891782837, -209.3591351345004341 ) ) ;
#20817=CARTESIAN_POINT ( 'NONE',  ( -9.720893520471410199, -287.4941441396226196, -341.8110988145703004 ) ) ;
#20818=CARTESIAN_POINT ( 'NONE',  ( 22.40417680613827045, -283.0044226538180965, -318.6994661230260135 ) ) ;
#20819=CARTESIAN_POINT ( 'NONE',  ( -113.0752690445126376, -284.8710785474981435, -284.2164490515212947 ) ) ;
#20820=CARTESIAN_POINT ( 'NONE',  ( 35.70285155340491201, -281.7313722969014407, -271.3116399768088058 ) ) ;
#20824=CARTESIAN_POINT ( 'NONE',  ( -90.71135064313021701, -291.6590203382359618, -324.2120837381959859 ) ) ;
#20825=CARTESIAN_POINT ( 'NONE',  ( -47.66019399952322289, -290.6085495531888228, -194.4998400290960774 ) ) ;
#20826=CARTESIAN_POINT ( 'NONE',  ( -93.95264491281066910, -272.2671482226831472, -223.8806758915478952 ) ) ;
#20827=CARTESIAN_POINT ( 'NONE',  ( 15.40273597902006131, -293.6783901606851259, -326.3194707647933797 ) ) ;
#20828=CARTESIAN_POINT ( 'NONE',  ( -76.25108930946325358, -288.0625010808399225, -332.9451989097763658 ) ) ;
#20829=CARTESIAN_POINT ( 'NONE',  ( 27.12809868588586681, -291.2999926311069885, -233.9023377423723957 ) ) ;
#20830=CARTESIAN_POINT ( 'NONE',  ( 26.70641927683401207, -288.2682997489649210, -234.4107056613696614 ) ) ;
#20831=CARTESIAN_POINT ( 'NONE',  ( -85.28047601435908120, -292.1948066931273615, -330.5268031993605859 ) ) ;
#20832=CARTESIAN_POINT ( 'NONE',  ( -105.4550436317330764, -292.9660349834684325, -238.8434519815604062 ) ) ;
#20833=CARTESIAN_POINT ( 'NONE',  ( -109.8572355757293906, -288.8064335118996269, -250.5253350984313272 ) ) ;
#20834=CARTESIAN_POINT ( 'NONE',  ( -94.45811135570875194, -293.2253713033337590, -221.7338168028446148 ) ) ;
#20835=CARTESIAN_POINT ( 'NONE',  ( -81.63036289327303052, -286.3734245513336987, -212.0351135088597232 ) ) ;
#20836=CARTESIAN_POINT ( 'NONE',  ( 31.63177611316188376, -295.1622739673917408, -240.4832332030868542 ) ) ;
#20837=CARTESIAN_POINT ( 'NONE',  ( -114.0814599542016055, -271.5444506490974277, -270.3482875283361295 ) ) ;
#20838=CARTESIAN_POINT ( 'NONE',  ( -82.61252422152907116, -275.4173829585836870, -210.0549499711476074 ) ) ;
#20839=CARTESIAN_POINT ( 'NONE',  ( -7.727338375026176820, -280.6638689043281261, -339.2667797889253620 ) ) ;
#20840=CARTESIAN_POINT ( 'NONE',  ( -81.78664796669242776, -294.8373789485053180, -333.1062935041177298 ) ) ;
#20841=CARTESIAN_POINT ( 'NONE',  ( -54.42395768749048557, -272.0695322114916621, -198.3460467296720253 ) ) ;
#20842=CARTESIAN_POINT ( 'NONE',  ( -94.73153460467943887, -275.9727444448810161, -317.7912353738931870 ) ) ;
#20843=CARTESIAN_POINT ( 'NONE',  ( -94.00444279580118234, -298.5265294166450190, -223.5379345244646458 ) ) ;
#20844=CARTESIAN_POINT ( 'NONE',  ( 36.02526616560538031, -273.8549504354530200, -248.8243745535157530 ) ) ;
#20845=CARTESIAN_POINT ( 'NONE',  ( -109.0553079769267839, -298.1934588575022076, -253.8525332928154796 ) ) ;
#20847=CARTESIAN_POINT ( 'NONE',  ( -105.1076338115589124, -296.9864173394244062, -297.9361058983351427 ) ) ;
#20849=CARTESIAN_POINT ( 'NONE',  ( 6.605588592710036622, -284.6659594329059360, -209.0837433538838184 ) ) ;
#20850=CARTESIAN_POINT ( 'NONE',  ( -63.07946570484787685, -297.7075374107682819, -201.9953597351392318 ) ) ;
#20851=CARTESIAN_POINT ( 'NONE',  ( -0.9695574409687663930, -286.5214441691337015, -202.4931046305520681 ) ) ;
#20852=CARTESIAN_POINT ( 'NONE',  ( 28.88339296018956404, -287.7302878641962707, -309.6037139327642649 ) ) ;
#20853=CARTESIAN_POINT ( 'NONE',  ( -112.6934909867121490, -298.5412128329006123, -269.6438912791250004 ) ) ;
#20854=CARTESIAN_POINT ( 'NONE',  ( -25.95290673324288377, -292.9066093389956791, -344.3227553983004441 ) ) ;
#20855=CARTESIAN_POINT ( 'NONE',  ( -92.94981500799279672, -278.4765414177834373, -217.2577905456915062 ) ) ;
#20856=CARTESIAN_POINT ( 'NONE',  ( -95.95921662488163406, -282.6952119285918457, -223.5744983911110353 ) ) ;
#20858=CARTESIAN_POINT ( 'NONE',  ( 23.83200740056147637, -286.9071004384716161, -310.9415329595228741 ) ) ;
#20860=CARTESIAN_POINT ( 'NONE',  ( 2.348985582641040626, -286.5201396420990818, -333.9979792785127302 ) ) ;
#20861=CARTESIAN_POINT ( 'NONE',  ( -35.81499124644425791, -299.6717045007252977, -196.5606880296625150 ) ) ;
#20862=CARTESIAN_POINT ( 'NONE',  ( -74.73554353817104356, -280.9897158211193187, -203.7254911128403307 ) ) ;
#20863=CARTESIAN_POINT ( 'NONE',  ( -110.9875180258348450, -294.7769342965548276, -254.3416535049790070 ) ) ;
#20864=CARTESIAN_POINT ( 'NONE',  ( 29.31445927877850366, -281.9544478712251134, -300.2502529616966171 ) ) ;
#20865=CARTESIAN_POINT ( 'NONE',  ( -113.2035059311331935, -296.5500998639170120, -283.8527604264756974 ) ) ;
#20866=CARTESIAN_POINT ( 'NONE',  ( -41.93067324659531181, -299.5133995266389775, -196.8108013356921902 ) ) ;
#20868=CARTESIAN_POINT ( 'NONE',  ( 36.69767369867167162, -283.7069798679340806, -282.4069486354017613 ) ) ;
#20869=CARTESIAN_POINT ( 'NONE',  ( -86.24854588009516476, -296.4121609665739356, -215.8493863450990773 ) ) ;
#20872=CARTESIAN_POINT ( 'NONE',  ( 15.09774189537612266, -284.2881463440410812, -323.5559644895413385 ) ) ;
#20874=CARTESIAN_POINT ( 'NONE',  ( 39.58706461736021254, -285.0523547857346784, -270.3937649182068981 ) ) ;
#20875=CARTESIAN_POINT ( 'NONE',  ( 24.23211951927487817, -275.3620944536096999, -316.3265784392799560 ) ) ;
#20876=CARTESIAN_POINT ( 'NONE',  ( 34.48355572900142363, -293.2124890900710739, -257.2481084673755731 ) ) ;
#20877=CARTESIAN_POINT ( 'NONE',  ( 32.01363576934313926, -283.4026846541706846, -295.4228514966454213 ) ) ;
#20878=CARTESIAN_POINT ( 'NONE',  ( 25.95156454694661008, -276.6347061329499297, -232.3095360414971253 ) ) ;
#20879=CARTESIAN_POINT ( 'NONE',  ( -96.70307339674830871, -285.3269018771783294, -318.4943923195729099 ) ) ;
#20880=CARTESIAN_POINT ( 'NONE',  ( 10.15402573352566051, -281.1753108169779125, -326.3858425914673944 ) ) ;
#20881=CARTESIAN_POINT ( 'NONE',  ( -94.63404593460406034, -281.2219457813750978, -221.9410674431646271 ) ) ;
#20882=CARTESIAN_POINT ( 'NONE',  ( -104.2305826856863433, -273.2154371772530226, -232.1112541988979103 ) ) ;
#20883=CARTESIAN_POINT ( 'NONE',  ( 30.54206305521553944, -275.8564585850491540, -306.8164333988646604 ) ) ;
#20884=CARTESIAN_POINT ( 'NONE',  ( 37.08266507870625617, -295.5132587783598979, -273.5262827114689230 ) ) ;
#20888=CARTESIAN_POINT ( 'NONE',  ( -111.1087109149389960, -294.4713458284537069, -287.7012183247330768 ) ) ;
#20890=CARTESIAN_POINT ( 'NONE',  ( -36.72926060950825899, -273.5677027891699140, -197.2897205765402475 ) ) ;
#20891=CARTESIAN_POINT ( 'NONE',  ( 38.54967042548561551, -295.1787554741550821, -278.7987952378402383 ) ) ;
#20892=CARTESIAN_POINT ( 'NONE',  ( 29.23719464318176620, -295.2529543887138743, -308.3531286958000805 ) ) ;
#20893=CARTESIAN_POINT ( 'NONE',  ( 35.49114571992429035, -289.7734966724760284, -287.5484678839014236 ) ) ;
#20894=CARTESIAN_POINT ( 'NONE',  ( -72.53843986620150019, -275.5189877936258540, -336.4150918836038500 ) ) ;
#20895=CARTESIAN_POINT ( 'NONE',  ( 14.75626865719569913, -278.2319686839630890, -323.6035608671764976 ) ) ;
#20896=CARTESIAN_POINT ( 'NONE',  ( -110.4554868740314646, -294.8138405551773076, -256.3044777016045259 ) ) ;
#20897=CARTESIAN_POINT ( 'NONE',  ( 37.95243297095561275, -283.2995713388204990, -261.4709942221876418 ) ) ;
#20898=CARTESIAN_POINT ( 'NONE',  ( -35.91371754338383226, -284.9908065015312673, -197.0659139083344371 ) ) ;
#20899=CARTESIAN_POINT ( 'NONE',  ( 105.0235304841314559, 114.7859377953624858, -281.8760858939756417 ) ) ;
#20901=CARTESIAN_POINT ( 'NONE',  ( -85.73698815178835275, -285.0271910793953793, -215.6127974910766056 ) ) ;
#20902=CARTESIAN_POINT ( 'NONE',  ( 35.32065431153155544, -282.9438863643317745, -295.0553005351545153 ) ) ;
#20904=CARTESIAN_POINT ( 'NONE',  ( -110.7319923787162708, -283.0696657928144191, -292.3583210136864636 ) ) ;
#20905=CARTESIAN_POINT ( 'NONE',  ( -86.66274888914290386, -280.3274454312755779, -211.4678977715739450 ) ) ;
#20908=CARTESIAN_POINT ( 'NONE',  ( -84.42324187753636977, -279.2066402739680484, -330.4785258047362504 ) ) ;
#20909=CARTESIAN_POINT ( 'NONE',  ( -21.33282851196159058, -297.3376638359844719, -340.3538533559490702 ) ) ;
#20910=CARTESIAN_POINT ( 'NONE',  ( 204.5909265758117783, 295.1816420246624944, -54.00000000003019096 ) ) ;
#20912=CARTESIAN_POINT ( 'NONE',  ( -110.3285070359494853, -274.7649140686125406, -253.8397848411426594 ) ) ;
#20913=CARTESIAN_POINT ( 'NONE',  ( -3.581603521288127645, -278.5200243446983563, -203.7728729229347664 ) ) ;
#20914=CARTESIAN_POINT ( 'NONE',  ( -111.9345783728541761, -292.4967461168567979, -255.8061178496796515 ) ) ;
#20915=CARTESIAN_POINT ( 'NONE',  ( 1.617149468239181820, -293.8651663714132951, -332.2765475686803711 ) ) ;
#20916=CARTESIAN_POINT ( 'NONE',  ( -103.7484836467933746, -289.5525222358883752, -309.3209310175312794 ) ) ;
#20918=CARTESIAN_POINT ( 'NONE',  ( 24.39937915826459758, -292.7292676166636625, -315.4014300198842875 ) ) ;
#20919=CARTESIAN_POINT ( 'NONE',  ( -72.74002389682556213, -283.9749907883933702, -205.5902876120702842 ) ) ;
#20920=CARTESIAN_POINT ( 'NONE',  ( -32.09321001925210481, -293.9794481883918138, -196.2988490738038365 ) ) ;
#20921=CARTESIAN_POINT ( 'NONE',  ( -74.02853751089649847, -284.8652946725479183, -334.1004946108089939 ) ) ;
#20923=CARTESIAN_POINT ( 'NONE',  ( -34.97969836027586865, -293.0223524817867542, -193.6196484299239273 ) ) ;
#20924=CARTESIAN_POINT ( 'NONE',  ( 4.953682423873231322, -281.1336348153731137, -210.7868865038511785 ) ) ;
#20925=CARTESIAN_POINT ( 'NONE',  ( -24.98705582815863124, -293.6930045112302423, -346.0149791639322530 ) ) ;
#20926=CARTESIAN_POINT ( 'NONE',  ( 19.51166936137877883, -289.0591087946734206, -322.0706911991779293 ) ) ;
#20927=CARTESIAN_POINT ( 'NONE',  ( -60.00316417309279871, -289.8305322261256833, -343.8865214185864829 ) ) ;
#20928=CARTESIAN_POINT ( 'NONE',  ( 23.53289057147818752, -287.1587408663851875, -229.9796017682292302 ) ) ;
#20931=CARTESIAN_POINT ( 'NONE',  ( 32.29085992876478173, -295.8005927074665351, -300.3535846594114105 ) ) ;
#20932=CARTESIAN_POINT ( 'NONE',  ( -36.17678014040627232, -296.7512821218360841, -193.8545191211221947 ) ) ;
#20934=CARTESIAN_POINT ( 'NONE',  ( -83.16328309463075641, -276.7559123518670390, -327.5559923027261107 ) ) ;
#20935=CARTESIAN_POINT ( 'NONE',  ( -63.53025098054684605, -273.2274431866519535, -198.0168942503060805 ) ) ;
#20936=CARTESIAN_POINT ( 'NONE',  ( -8.981782967233312931, -293.1542597173978493, -338.3926640260614818 ) ) ;
#20937=CARTESIAN_POINT ( 'NONE',  ( 20.63548272896129276, -276.6715377598141004, -224.3341054917140411 ) ) ;
#20938=CARTESIAN_POINT ( 'NONE',  ( -55.52117181844066351, -296.0549884609121136, -198.5621394372791144 ) ) ;
#20939=CARTESIAN_POINT ( 'NONE',  ( 33.13573248648712877, -295.0274081169410465, -290.9017386271651162 ) ) ;
#20940=CARTESIAN_POINT ( 'NONE',  ( -68.63685933805450645, -296.5530192012665793, -336.6684889897231869 ) ) ;
#20942=CARTESIAN_POINT ( 'NONE',  ( -101.5627680980408769, -294.0295443666564665, -309.4211084301740584 ) ) ;
#20943=CARTESIAN_POINT ( 'NONE',  ( -107.9332090816532599, -273.7438928579061326, -239.8785732479233559 ) ) ;
#20944=CARTESIAN_POINT ( 'NONE',  ( 10.48454465268249791, -286.9515741042035870, -326.3572326024889776 ) ) ;
#20945=CARTESIAN_POINT ( 'NONE',  ( -112.1864798006810275, -274.6238543444303559, -264.7895706816638040 ) ) ;
#20946=CARTESIAN_POINT ( 'NONE',  ( -60.85827982244397560, -274.2474350844931337, -197.0491494324768098 ) ) ;
#20947=CARTESIAN_POINT ( 'NONE',  ( -107.4808590807963071, -297.1540169585817353, -250.0489081515501084 ) ) ;
#20948=CARTESIAN_POINT ( 'NONE',  ( -35.40414227653018742, -282.0562151002807241, -195.0179709589839092 ) ) ;
#20949=CARTESIAN_POINT ( 'NONE',  ( 27.44274510741312056, -279.6995619370768509, -229.5644554990647066 ) ) ;
#20951=CARTESIAN_POINT ( 'NONE',  ( 13.60703821590156082, -281.7093275045192513, -328.0300693289917149 ) ) ;
#20952=CARTESIAN_POINT ( 'NONE',  ( 24.40298689390812470, -274.2905066446334672, -224.5254723403164974 ) ) ;
#20953=CARTESIAN_POINT ( 'NONE',  ( -3.989172553448509184, -278.8845380209128280, -201.8336158705793935 ) ) ;
#20954=CARTESIAN_POINT ( 'NONE',  ( -5.692183963668587587, -278.4672254734427952, -202.1824075429152856 ) ) ;
#20955=CARTESIAN_POINT ( 'NONE',  ( -81.40946127837015922, -272.0145324676538507, -211.3615682054955585 ) ) ;
#20956=CARTESIAN_POINT ( 'NONE',  ( 26.85111234636556432, -278.0730929238549720, -309.2452779252170671 ) ) ;
#20959=CARTESIAN_POINT ( 'NONE',  ( -30.81407025375910536, -290.1542461436179678, -195.2375421658138066 ) ) ;
#20960=CARTESIAN_POINT ( 'NONE',  ( -67.01544435105675745, -291.6737943119039755, -199.3085395368101445 ) ) ;
#20961=B_SPLINE_CURVE_WITH_KNOTS ( 'NONE', 3,
 ( #44565, #66817, #66367, #53062, #9502, #65924, #15704, #29914, #74376, #89496, #46419, #81021, #73468, #16623, #8580, #45960, #38390, #24659, #74865, #73918, #81474, #1036, #1950, #81937, #37913, #59740, #2882, #23263, #67302, #9035, #30847, #1485, #9977, #2430, #58798, #17092, #45477, #88582, #60196, #53547, #30368, #89034, #24184, #67756, #31767, #60659, #23730, #82420, #37458, #59257, #17568, #87643, #52593, #8126, #45017, #22791, #51660, #80547, #88105, #52141, #75781, #61591, #68220, #90423, #33159, #10901, #54933, #12319, #41163, #55421, #68693, #26533, #84274, #11386, #19425, #70100, #19889, #62050, #90884, #75320, #39768, #47341, #18966, #26047, #69617, #55888, #5241, #40238, #83813, #34112, #33625, #3340, #47819, #63014, #39303, #83333, #91845, #61139, #3824, #10437, #27000, #76721, #32705, #69153, #48287, #11847, #40697, #32231, #62534, #84742, #18025, #4281, #25580, #77190, #4745, #89975, #82872, #25129, #91375, #54003, #46879, #54463, #18479, #76258, #86146, #27956, #57304, #70574, #12817, #5699, #87080, #34574, #41657, #48760, #35972, #64433, #78599, #64892, #57760, #63483, #56821, #13279, #50652, #21297, #77665, #28873, #50169, #13742, #71983, #456, #42116, #42591, #56846, #6166, #71506, #63949, #71032, #79066, #86606, #58236, #43535, #92314, #49703, #27468, #85687, #93259, #20834, #6639, #21776, #14218, #49246, #43078, #85224, #65349, #35519, #7101, #28413, #79540, #35035, #56361, #7549, #14679, #72432, #36434, #29343, #20375, #78141, #92788, #39071, #22229, #81705, #24898, #31537, #46647, #75549, #65817, #51099, #10673, #23952, #2658, #88805, #24415, #67984, #16854, #90204, #32474, #60425, #54233, #3110, #72883, #79986, #31993, #17337, #83102, #60885, #18255, #89736, #8008, #15123, #53778, #46188, #43986, #82645, #25353, #82181, #61820, #36900, #53295, #45709, #47108, #76015, #2195, #31079, #89265, #17794, #74622, #75093, #61371, #39528, #68449, #59967, #52827, #67528, #3584, #9751, #38625, #11148, #40010, #68927, #10202, #4058, #32928, #13510, #48523, #62288, #20611, #49481, #34343, #69853, #5473, #18729, #62782, #70347, #49013, #25813, #55655, #41889, #26770, #77424, #85464, #12085, #27236, #91615, #84508, #55189, #92545, #63250, #54693, #70800, #92081, #19654, #83567, #47590, #11617, #56124, #77911, #84977, #20128, #13053, #12563, #42359, #91124, #26295, #5935, #76494, #41414, #90652, #4987, #34807, #63720, #27713, #71272, #56612, #78371, #76957, #40462, #40933, #6399, #84047, #35271, #69380, #4512, #33389, #19193, #48052, #33873, #224, #44219, #58919, #8704, #22010, #64200, #28644, #65586, #72207, #87308, #22455, #13976, #93031, #51328, #64663, #43311, #35750, #30038, #93491, #36666, #7780, #58464, #14454, #49934, #57534, #28187, #36202, #701, #21529, #29104, #73127, #14904, #29585, #21066, #80221, #1155, #6877, #57998, #86378, #15359, #8254, #57076, #71751, #85915, #37135, #80679, #50880, #50409, #87767, #22919, #66043, #7324, #72659, #78830, #42834, #79315, #65121, #86854, #79762, #43759, #51789, #15835, #44692, #73593, #46544, #38524, #9637, #2086, #39430, #10104, #66493, #17694, #74993, #67428, #60785, #82999, #30976, #2556, #16749, #88705, #31435, #52719, #59864, #67883, #24791, #66947, #46086, #23400, #60325, #37582, #45604, #53190, #89162, #24312, #75447, #38972, #38039, #3007, #74042, #54128, #74506, #89623, #82068, #10565, #23853, #68347, #81601, #82543, #3474, #17224, #32365, #61266, #75908, #31892, #53676, #1610, #90101, #25252, #18151, #47004, #30495, #81146, #59389, #88241, #52266, #16290, #45143, #9160, #55549, #69277, #77794, #20015, #83941, #41782, #84398, #61714, #68822, #19547, #4875, #70693, #26660, #63141, #32824, #48413, #5823, #11976, #4406, #12944, #90548, #34235, #70234, #3952, #77316, #34697, #69743, #49371, #11033, #40824, #33285, #63610, #92434, #25706, #54589, #76849, #12450, #91970, #62180, #27598, #40360, #33759, #83460, #76389, #55072, #5368, #18616, #11513, #56495, #27125, #85354, #91013, #26181, #19094, #20502, #62670, #47947, #41298, #47480, #48893, #56008, #39901, #91504, #84864, #57881, #36552, #13402, #43201, #29469, #14342, #36092, #73009, #93382, #14797, #79199, #50293, #42717, #20956, #29925, #6766, #92918, #79656, #65469, #42246, #71159, #28080, #50771, #586, #43652, #86736, #72548, #72102, #1046, #78722, #13863, #21898, #64079, #71634, #78264, #7219, #37021, #58809, #35641, #87653, #7670, #80107, #64558, #6287, #28534, #65013, #57426, #58357, #15246, #44104, #87197, #86267, #22345, #22804, #28993, #85806, #51216, #35158, #21418, #113, #8138, #56968, #65935, #49825, #67310, #45969, #32240, #17578, #81483, #2440, #46427, #75330, #52602, #24193, #89043, #74875, #1964, #45027, #10445, #15715, #66825, #38401, #24670, #37921, #1495, #39311, #53070, #80562, #61148, #31318, #59270, #81945, #44577, #60205, #51671 ),
 .UNSPECIFIED., .F., .F.,
 ( 4, 1, 1, 1, 2, 2, 2, 2, 2, 2, 2, 2, 2, 2, 2, 2, 2, 2, 2, 2, 2, 2, 2, 2, 2, 2, 2, 2, 2, 2, 2, 2, 2, 2, 2, 2, 2, 2, 2, 2, 2, 2, 2, 2, 2, 2, 2, 2, 2, 2, 2, 2, 2, 2, 2, 2, 2, 2, 2, 2, 2, 2, 2, 2, 2, 2, 2, 2, 2, 2, 2, 2, 2, 2, 2, 2, 2, 2, 2, 2, 2, 2, 2, 2, 2, 2, 2, 2, 2, 2, 2, 2, 2, 2, 2, 2, 2, 2, 2, 2, 2, 2, 2, 2, 2, 2, 2, 2, 2, 2, 2, 2, 2, 2, 2, 2, 2, 2, 2, 2, 2, 2, 2, 2, 2, 2, 2, 2, 2, 2, 2, 2, 2, 2, 2, 2, 2, 2, 2, 2, 2, 2, 2, 2, 2, 2, 2, 2, 2, 2, 2, 2, 2, 2, 2, 2, 2, 2, 2, 2, 2, 2, 2, 2, 2, 2, 2, 2, 2, 2, 2, 2, 2, 2, 2, 2, 2, 2, 2, 2, 2, 2, 2, 2, 2, 2, 2, 2, 2, 2, 2, 2, 2, 2, 2, 2, 2, 2, 2, 2, 2, 2, 2, 2, 2, 2, 2, 2, 2, 2, 2, 2, 2, 2, 2, 2, 2, 2, 2, 2, 2, 2, 2, 2, 2, 2, 2, 2, 2, 2, 2, 2, 2, 2, 2, 2, 2, 2, 2, 2, 2, 2, 2, 2, 2, 2, 2, 2, 2, 2, 2, 2, 2, 2, 2, 2, 2, 2, 2, 2, 2, 2, 2, 2, 2, 2, 2, 2, 2, 2, 2, 2, 2, 2, 2, 2, 2, 2, 2, 2, 2, 2, 2, 2, 2, 2, 2, 2, 2, 2, 2, 2, 2, 2, 2, 2, 2, 2, 2, 2, 2, 2, 4 ),
 ( -0.05114157420909415386, -0.02298090003068697235, -0.008900562941483385060, -0.001860394396881591417, -0.0001003522607311430059, 0.0007796688073440846689, 0.001659689875419305405, 0.005179774147720181410, 0.008699858420021057415, 0.01221994269232193342, 0.01397998482847236101, 0.01574002696462277473, 0.01926011123692361604, 0.02278019550922444347, 0.02630027978152527091, 0.02806032191767569850, 0.02982036405382612609, 0.03334044832612698128, 0.03686053259842785035, 0.04038061687072870554, 0.04214065900687911925, 0.04390070114302953297, 0.04742078541533041591, 0.05094086968763129886, 0.05446095395993218180, 0.05622099609608263715, 0.05798103823223307862, 0.06150112250453390605, 0.06502120677683471961, 0.06854129104913554704, 0.07030133318528596076, 0.07206137532143638835, 0.07558145959373727130, 0.07910154386603812648, 0.08262162813833900943, 0.08438167027448945090, 0.08614171241063992013, 0.08966179668294077532, 0.09318188095524163050, 0.09670196522754251345, 0.09846200736369295492, 0.1002220494998433964, 0.1037421337721442793, 0.1072622180444451623, 0.1107823023167460175, 0.1143023865890469004, 0.1178224708613477834, 0.1213425551336486385, 0.1248626394059495215, 0.1283827236782504044, 0.1301427658144008181, 0.1319028079505512596, 0.1354228922228521148, 0.1389429764951529978, 0.1424630607674538807, 0.1442231029036042944, 0.1459831450397547081, 0.1495032293120556466, 0.1530233135843565850, 0.1565433978566575512, 0.1583034399928080482, 0.1600634821289586007, 0.1635835664012597057, 0.1671036506735608385, 0.1706237349458619434, 0.1723837770820125237, 0.1741438192181630762, 0.1776639034904642367, 0.1811839877627653972, 0.1847040720350665299, 0.1864641141712171102, 0.1882241563073677459, 0.1917442405796688787, 0.1952643248519700392, 0.1987844091242711719, 0.2005444512604217522, 0.2023044933965723602, 0.2058245776688735207, 0.2093446619411746812, 0.2128647462134758417, 0.2146247883496263942, 0.2163848304857770022, 0.2199049147580781627, 0.2234249990303793787, 0.2269450833026805947, 0.2287051254388311472, 0.2304651675749816997, 0.2339852518472829157, 0.2375053361195841317, 0.2410254203918853477, 0.2427854625280359002, 0.2445455046641863972, 0.2480655889364875022, 0.2515856732087886072, 0.2551057574810897122, 0.2568657996172403202, 0.2586258417533908172, 0.2621459260256919221, 0.2656660102979930271, 0.2691860945702941321, 0.2709461367064446846, 0.2727061788425952371, 0.2762262631148963421, 0.2797463473871973916, 0.2832664316594984966, 0.2850264737956491601, 0.2867865159317997126, 0.2903066002041009286, 0.2938266844764020891, 0.2973467687487033051, 0.2991068108848539131, 0.3008668530210045211, 0.3043869372933057371, 0.3079070215656068976, 0.3114271058379081136, 0.3131871479740586661, 0.3149471901102093296, 0.3184672743825104901, 0.3219873586548117061, 0.3255074429271129222, 0.3272674850632635302, 0.3290275271994141937, 0.3325476114717154652, 0.3360676957440166812, 0.3395877800163179527, 0.3413478221524685607, 0.3431078642886192243, 0.3466279485609204958, 0.3501480328332218228, 0.3536681171055230943, 0.3571882013778244214, 0.3607082856501256929, 0.3642283699224270199, 0.3677484541947282914, 0.3712685384670296185, 0.3730285806031802820, 0.3747886227393308900, 0.3783087070116322725, 0.3818287912839335996, 0.3853488755562349266, 0.3871089176923856456, 0.3888689598285362536, 0.3923890441008375807, 0.3959091283731389632, 0.3994292126454403458, 0.4011892547815910093, 0.4029492969177416173, 0.4064693811900430553, 0.4099894654623443824, 0.4135095497346458204, 0.4152695918707965395, 0.4170296340069470920, 0.4205497182792485300, 0.4240698025515499126, 0.4275898868238513506, 0.4293499289600020141, 0.4311099710961525666, 0.4346300553684539492, 0.4381501396407551652, 0.4416702239130565477, 0.4434302660492072112, 0.4451903081853577637, 0.4487103924576591463, 0.4522304767299604178, 0.4557505610022617448, 0.4575106031384122973, 0.4592706452745629608, 0.4627907295468641768, 0.4663108138191653929, 0.4698308980914666089, 0.4715909402276171614, 0.4733509823637678249, 0.4768710666360691519, 0.4803911509083702569, 0.4839112351806714729, 0.4856712773168221364, 0.4874313194529727999, 0.4909514037252741270, 0.4944714879975753430, 0.4979915722698766700, 0.4997516144060273335, 0.5015116565421779971, 0.5050317408144793241, 0.5085518250867805401, 0.5120719093590818671, 0.5138319514952325306, 0.5155919936313831942, 0.5191120779036842992, 0.5226321621759855152, 0.5261522464482867312, 0.5279122885844372837, 0.5296723307205878362, 0.5331924149928890522, 0.5367124992651902682, 0.5402325835374913732, 0.5419926256736420367, 0.5437526678097925892, 0.5472727520820938052, 0.5507928363543951322, 0.5543129206266964593, 0.5560729627628470118, 0.5578330048989975642, 0.5613530891712987803, 0.5648731734436001073, 0.5683932577159014343, 0.5701532998520520978, 0.5719133419882027614, 0.5754334262605039774, 0.5789535105328053044, 0.5824735948051066314, 0.5842336369412572949, 0.5859936790774079585, 0.5895137633497090635, 0.5930338476220103905, 0.5965539318943114955, 0.6000740161666127115, 0.6035941004389139275, 0.6071141847112151435, 0.6106342689835162485, 0.6141543532558175755, 0.6159143953919681280, 0.6176744375281187915, 0.6211945218004200076, 0.6247146060727212236, 0.6282346903450223286, 0.6299947324811729921, 0.6317547746173236556, 0.6352748588896248716, 0.6387949431619260876, 0.6423150274342271926, 0.6440750695703779671, 0.6458351117065286306, 0.6493551959788298467, 0.6528752802511311737, 0.6563953645234323897, 0.6581554066595831642, 0.6599154487957338278, 0.6634355330680350438, 0.6669556173403363708, 0.6704757016126375868, 0.6722357437487883614, 0.6739957858849390249, 0.6775158701572402409, 0.6810359544295415679, 0.6845560387018427839, 0.6863160808379935585, 0.6880761229741442220, 0.6915962072464454380, 0.6951162915187467650, 0.6986363757910479810, 0.7003964179271987556, 0.7021564600633494191, 0.7056765443356506351, 0.7091966286079519621, 0.7127167128802531781, 0.7144767550164039527, 0.7162367971525546162, 0.7197568814248558322, 0.7232769656971571592, 0.7267970499694583753, 0.7285570921056091498, 0.7303171342417598133, 0.7338372185140609183, 0.7373573027863620233, 0.7408773870586633503, 0.7426374291948140138, 0.7443974713309645663, 0.7479175556032657823, 0.7514376398755669983, 0.7549577241478682144, 0.7567177662840187669, 0.7584778084201693193, 0.7619978926924704243, 0.7655179769647714183, 0.7690380612370726343, 0.7707981033732231868, 0.7725581455093736283, 0.7760782297816749553, 0.7795983140539760603, 0.7831183983262772763, 0.7848784404624279398, 0.7866384825985783813, 0.7901585668708795973, 0.7936786511431808133, 0.7971987354154820293, 0.7989587775516325818, 0.8007188196877832453, 0.8042389039600844614, 0.8077589882323856774, 0.8112790725046868934, 0.8130391146408373348, 0.8147991567769879984, 0.8183192410492892144, 0.8218393253215903194, 0.8253594095938916464, 0.8271194517300421989, 0.8288794938661928624, 0.8323995781384940784, 0.8359196624107952944, 0.8394397466830965104, 0.8429598309553976154, 0.8464799152276989425, 0.8499999995000000474 ),
 .UNSPECIFIED. ) ;
#20962=CARTESIAN_POINT ( 'NONE',  ( 37.55594080225193210, -277.6337173120213038, -276.7149992892133810 ) ) ;
#20963=CARTESIAN_POINT ( 'NONE',  ( -4.407434547962546745, -272.4859908285420147, -202.9649056997094476 ) ) ;
#20966=CARTESIAN_POINT ( 'NONE',  ( -108.2114402159723028, -282.8714997662547148, -245.6595842048252791 ) ) ;
#20968=CARTESIAN_POINT ( 'NONE',  ( 1.768504347131608645, -293.3115930758016816, -332.5302597307751853 ) ) ;
#20969=CARTESIAN_POINT ( 'NONE',  ( 24.52604001798687250, -286.2518659473237221, -311.4117337935249452 ) ) ;
#20972=CARTESIAN_POINT ( 'NONE',  ( -31.47052432468297312, -292.9779849412669250, -345.1824508631195272 ) ) ;
#20973=CARTESIAN_POINT ( 'NONE',  ( -105.1767457852696026, -282.5762602560212144, -305.4209095206774691 ) ) ;
#20974=CARTESIAN_POINT ( 'NONE',  ( -106.2686978920281291, -280.5023525591585098, -243.8453675696348171 ) ) ;
#20975=CARTESIAN_POINT ( 'NONE',  ( -113.9572554671480162, -285.7259166477047643, -272.8517141236003454 ) ) ;
#20976=CARTESIAN_POINT ( 'NONE',  ( 37.66393624701710507, -279.9472852888584953, -282.6130566177410515 ) ) ;
#20977=CARTESIAN_POINT ( 'NONE',  ( 24.95072229601622027, -287.0277528565018770, -232.2999289767265054 ) ) ;
#20978=CARTESIAN_POINT ( 'NONE',  ( -48.68086744841769331, -278.6245043657041265, -343.1232920335880863 ) ) ;
#20979=CARTESIAN_POINT ( 'NONE',  ( -78.71491368497885333, -278.4279185479413741, -330.7623315307636744 ) ) ;
#20980=CARTESIAN_POINT ( 'NONE',  ( -99.65097874842462033, -287.1041281900666604, -227.8901231934778195 ) ) ;
#20982=CARTESIAN_POINT ( 'NONE',  ( -105.2526074958591806, -296.8557454040462176, -233.9560239301554816 ) ) ;
#20983=CARTESIAN_POINT ( 'NONE',  ( -2.578389189232592749, -290.5703104147995077, -336.4741027412723042 ) ) ;
#20985=CARTESIAN_POINT ( 'NONE',  ( -119.3990491898856732, -287.0519495502701943, -270.3937649182068412 ) ) ;
#20987=CARTESIAN_POINT ( 'NONE',  ( -57.60236806042784252, -271.7911514786489988, -197.9223941613907698 ) ) ;
#20988=CARTESIAN_POINT ( 'NONE',  ( 25.84110480896405804, -291.3838489219122039, -227.6727997809887256 ) ) ;
#20989=CARTESIAN_POINT ( 'NONE',  ( -105.0212628728115476, -295.6914460922606622, -297.8832041714238130 ) ) ;
#20990=CARTESIAN_POINT ( 'NONE',  ( 33.32942174276556813, -288.7979529030894241, -249.4288412032416602 ) ) ;
#20991=PRODUCT ( 'High-Pressure Air Hose', 'High-Pressure Air Hose', '', ( #24624 ) ) ;
#20992=CARTESIAN_POINT ( 'NONE',  ( 33.70105190369956460, -283.0414435020989572, -249.6029533667195324 ) ) ;
#20993=CARTESIAN_POINT ( 'NONE',  ( -99.38116766687564052, -291.3813436920794402, -314.9897021226811944 ) ) ;
#20994=CARTESIAN_POINT ( 'NONE',  ( -110.3064229726024763, -291.5743301758000143, -293.5437952325392530 ) ) ;
#20995=CARTESIAN_POINT ( 'NONE',  ( -84.02010819400756247, -285.6932732885861128, -329.1314622496981315 ) ) ;
#20996=CARTESIAN_POINT ( 'NONE',  ( -54.12918068643331537, -277.4285212899328030, -345.5634825142376485 ) ) ;
#20998=CARTESIAN_POINT ( 'NONE',  ( -63.78556762282077131, -293.4741203252553987, -341.1427262545600456 ) ) ;
#20999=CARTESIAN_POINT ( 'NONE',  ( 31.07617318620259539, -281.8408462702693100, -305.6880852403859876 ) ) ;
#21000=CARTESIAN_POINT ( 'NONE',  ( -40.85674713035532335, -275.8680216950203885, -196.1586392236647498 ) ) ;
#21001=CARTESIAN_POINT ( 'NONE',  ( 39.58706461736021254, -290.0519495502703080, -270.3284710469133074 ) ) ;
#21002=CARTESIAN_POINT ( 'NONE',  ( 37.22868403769292911, -273.6069568449494795, -255.7586585530844445 ) ) ;
#21004=CARTESIAN_POINT ( 'NONE',  ( 22.16725555787966684, -280.4681939593478432, -227.9739426233922188 ) ) ;
#21005=CARTESIAN_POINT ( 'NONE',  ( -113.6498229292669606, -279.8489205516154925, -263.0670781371906060 ) ) ;
#21006=CARTESIAN_POINT ( 'NONE',  ( -100.4110810367438091, -298.4961095583690849, -232.3459152040091737 ) ) ;
#21007=CARTESIAN_POINT ( 'NONE',  ( -16.21812605038069321, -281.8444377094382958, -344.2174164699054586 ) ) ;
#21008=CARTESIAN_POINT ( 'NONE',  ( -110.7076259378346208, -292.4443482789500308, -260.2120705860857584 ) ) ;
#21009=CARTESIAN_POINT ( 'NONE',  ( -67.24071266760248022, -275.2667106382818361, -200.2719642868421488 ) ) ;
#21010=CARTESIAN_POINT ( 'NONE',  ( -80.98291549295413461, -274.7886540384796490, -207.4578900942628650 ) ) ;
#21012=CARTESIAN_POINT ( 'NONE',  ( -7.227749053095210208, -296.6564308410267472, -338.8818150961515130 ) ) ;
#21013=CARTESIAN_POINT ( 'NONE',  ( -97.40816235265968714, -281.9413254738955175, -314.9934890276267083 ) ) ;
#21014=CARTESIAN_POINT ( 'NONE',  ( -68.31636199602947102, -291.3230275388935411, -199.8746715106072998 ) ) ;
#21015=CARTESIAN_POINT ( 'NONE',  ( 8.572711529114068085, -274.4402099682191647, -329.2802861744372080 ) ) ;
#21016=CARTESIAN_POINT ( 'NONE',  ( -3.859450391070875064, -288.0865563404634031, -201.8969122317749907 ) ) ;
#21017=CARTESIAN_POINT ( 'NONE',  ( -93.66855322616524404, -290.1355808120229085, -223.4212561549220766 ) ) ;
#21019=CARTESIAN_POINT ( 'NONE',  ( -113.8007302467491542, -289.1162581910467111, -271.2040025293756571 ) ) ;
#21020=CARTESIAN_POINT ( 'NONE',  ( -98.86186408727481023, -289.6749262385654333, -309.6975757944746874 ) ) ;
#21022=CARTESIAN_POINT ( 'NONE',  ( 36.49057284273963830, -288.8933597157793542, -291.1526935178251847 ) ) ;
#21023=CARTESIAN_POINT ( 'NONE',  ( 17.45390565889626444, -276.5746131182507952, -318.6451781088040889 ) ) ;
#21024=CARTESIAN_POINT ( 'NONE',  ( 13.18181335384396391, -293.2858785741150882, -328.1278525517369644 ) ) ;
#21025=CARTESIAN_POINT ( 'NONE',  ( -58.45079190907373601, -283.9693619512170812, -344.3605674878631930 ) ) ;
#21026=CARTESIAN_POINT ( 'NONE',  ( -91.89100066589773519, -285.6326949933856554, -216.0461283174732614 ) ) ;
#21028=CARTESIAN_POINT ( 'NONE',  ( 17.62357177023229937, -282.5711191151791581, -318.4330055258355969 ) ) ;
#21029=CARTESIAN_POINT ( 'NONE',  ( -56.32961566068995296, -169.3491268111188219, -364.4629006607140127 ) ) ;
#21030=CARTESIAN_POINT ( 'NONE',  ( 198.4191458182635017, 289.3439720879956099, -97.25198484077063199 ) ) ;
#21031=CARTESIAN_POINT ( 'NONE',  ( -112.1541305756452402, -270.5365672045004430, -270.3354547578530287 ) ) ;
#21032=CARTESIAN_POINT ( 'NONE',  ( -62.07469003415040731, -272.9193124220362847, -201.5070626395322790 ) ) ;
#21033=CARTESIAN_POINT ( 'NONE',  ( -36.71969321418954024, -272.9804737547783589, -197.0421757620138123 ) ) ;
#21034=CARTESIAN_POINT ( 'NONE',  ( -19.30779366272476949, -294.3339289529244525, -345.2110462503962367 ) ) ;
#21035=CARTESIAN_POINT ( 'NONE',  ( -87.69934636623491997, -230.2613027696342840, -344.8992764788239356 ) ) ;
#21036=CARTESIAN_POINT ( 'NONE',  ( -36.92548852504683765, -272.7421257071342779, -193.8424301553349949 ) ) ;
#21037=CARTESIAN_POINT ( 'NONE',  ( -35.80686752662442274, -299.9319789466649127, -196.1254176205127067 ) ) ;
#21038=CARTESIAN_POINT ( 'NONE',  ( 1.586900746562427189, -289.8349396974593333, -332.6973635512485430 ) ) ;
#21039=CARTESIAN_POINT ( 'NONE',  ( -110.5552296144252438, -291.6926677895818329, -265.7297335455925804 ) ) ;
#21041=CARTESIAN_POINT ( 'NONE',  ( -112.9096099239331039, -297.6627823977966614, -256.8588506751494833 ) ) ;
#21042=CARTESIAN_POINT ( 'NONE',  ( 29.48388025221274944, -288.4431397842553793, -300.0219005406169686 ) ) ;
#21043=CARTESIAN_POINT ( 'NONE',  ( 24.76181545558662123, -294.9570124622788398, -315.6305189611206856 ) ) ;
#21044=CARTESIAN_POINT ( 'NONE',  ( -36.26901294854877023, -295.5314227784099899, -347.3051948174285712 ) ) ;
#21045=CARTESIAN_POINT ( 'NONE',  ( 35.42460380009403309, -293.7958266790826087, -276.1976423869222117 ) ) ;
#21047=CARTESIAN_POINT ( 'NONE',  ( 24.14068485488863658, -276.8791087063765985, -226.4159862955499420 ) ) ;
#21050=CARTESIAN_POINT ( 'NONE',  ( -91.01074608189379944, -278.8225538302208975, -215.1582707267325532 ) ) ;
#21051=CARTESIAN_POINT ( 'NONE',  ( 20.49504038287555119, -273.3118124547708589, -224.5003849545063304 ) ) ;
#21052=CARTESIAN_POINT ( 'NONE',  ( 20.03237936985398449, -275.8527811600368409, -224.8259661269908065 ) ) ;
#21053=CARTESIAN_POINT ( 'NONE',  ( -24.35513660618481779, -275.9757496940782175, -195.4389608324812002 ) ) ;
#21054=CARTESIAN_POINT ( 'NONE',  ( 37.29853088105747361, -273.4399196808178090, -260.0053119979341432 ) ) ;
#21055=CARTESIAN_POINT ( 'NONE',  ( -82.01295401248555095, -298.0764271405614068, -212.4318408627218275 ) ) ;
#21056=CARTESIAN_POINT ( 'NONE',  ( -110.8310390908306573, -295.0767137119880772, -274.1941291371088028 ) ) ;
#21058=CARTESIAN_POINT ( 'NONE',  ( -104.7426967551842978, -279.5254439140075533, -233.2581186867105032 ) ) ;
#21059=CARTESIAN_POINT ( 'NONE',  ( -45.90599148361290105, -277.3303090215767384, -342.9076257397211975 ) ) ;
#21060=CARTESIAN_POINT ( 'NONE',  ( 36.90234632908327939, -286.0044285509882229, -251.8916881014038438 ) ) ;
#21061=CARTESIAN_POINT ( 'NONE',  ( -109.8903953936069513, -274.7990515606630879, -251.1440210749231596 ) ) ;
#21062=CARTESIAN_POINT ( 'NONE',  ( 82.64408888120264862, -299.9321935367201490, -197.8381816864644520 ) ) ;
#21063=CARTESIAN_POINT ( 'NONE',  ( 33.23496061135709567, -287.0056384659935134, -289.8243024082034367 ) ) ;
#21064=CARTESIAN_POINT ( 'NONE',  ( 5.528082745358883443, -278.8815090242043766, -210.0274148995039809 ) ) ;
#21065=CARTESIAN_POINT ( 'NONE',  ( -7.745948802577005132, -279.0225108815593558, -202.9717709099863328 ) ) ;
#21066=CARTESIAN_POINT ( 'NONE',  ( -67.46184869737096790, -285.4473543557164703, -339.0610184254437627 ) ) ;
#21067=CARTESIAN_POINT ( 'NONE',  ( 15.89640231059415854, -277.4815847903368535, -320.8867051006063775 ) ) ;
#21069=CARTESIAN_POINT ( 'NONE',  ( -5.727086149433370466, -274.8819777967572691, -339.4588039038982288 ) ) ;
#21070=CARTESIAN_POINT ( 'NONE',  ( 20.75750026452003283, -275.5802556465244493, -225.9741374621141574 ) ) ;
#21071=CARTESIAN_POINT ( 'NONE',  ( 35.54709598299938023, -283.3169278434688749, -251.9967004419412149 ) ) ;
#21073=CARTESIAN_POINT ( 'NONE',  ( 35.75763782286033177, -289.7162696096799550, -289.4870425833998979 ) ) ;
#21074=CARTESIAN_POINT ( 'NONE',  ( 25.08619535696503178, -292.1138942037821380, -311.9504398847830657 ) ) ;
#21075=CARTESIAN_POINT ( 'NONE',  ( 82.15506381819601245, -299.0670410310526108, -197.3076072666646326 ) ) ;
#21076=CARTESIAN_POINT ( 'NONE',  ( -68.47635553081295257, -272.3191494584230554, -203.7749868104250197 ) ) ;
#21077=CARTESIAN_POINT ( 'NONE',  ( 36.13362775344320710, -291.5542996729639640, -259.7667009052776166 ) ) ;
#21078=CARTESIAN_POINT ( 'NONE',  ( 89.65909921107042635, 79.73535476480827811, -300.8268380169218972 ) ) ;
#21080=CARTESIAN_POINT ( 'NONE',  ( -69.08668196632139313, -287.9419974301690104, -339.7653544813170470 ) ) ;
#21081=CARTESIAN_POINT ( 'NONE',  ( -65.60341423208502931, -285.0281113846423864, -338.5490225238742710 ) ) ;
#21082=CARTESIAN_POINT ( 'NONE',  ( 11.44437779676107780, -284.9573874184537772, -212.0353161358927423 ) ) ;
#21083=CARTESIAN_POINT ( 'NONE',  ( -42.95993448864535225, -284.5495851033617214, -343.7860621014394269 ) ) ;
#21084=CARTESIAN_POINT ( 'NONE',  ( -109.6563736073138244, -285.2046216848851259, -281.7849389376270892 ) ) ;
#21085=CARTESIAN_POINT ( 'NONE',  ( -91.64468435172817351, -293.2635032283860141, -218.0413508963960112 ) ) ;
#21087=CARTESIAN_POINT ( 'NONE',  ( 30.55047328220840441, -274.0673387295746011, -303.6459637433583225 ) ) ;
#21088=CARTESIAN_POINT ( 'NONE',  ( -44.04514827787810560, -274.3030101501432796, -193.6213972867191444 ) ) ;
#21089=CARTESIAN_POINT ( 'NONE',  ( -93.62209232859034103, -289.3289734142277894, -219.9445368509293246 ) ) ;
#21090=CARTESIAN_POINT ( 'NONE',  ( 14.88317882177516971, -276.3404187383079602, -327.0160342192095300 ) ) ;
#21091=CARTESIAN_POINT ( 'NONE',  ( 31.00599725859574107, -295.9268299466259577, -300.3684347852315000 ) ) ;
#21093=CARTESIAN_POINT ( 'NONE',  ( 35.77081079830085031, -295.8376638359844719, -253.6410175316879361 ) ) ;
#21094=CARTESIAN_POINT ( 'NONE',  ( -106.9943554979259801, -283.5482330340972226, -246.7551050580815968 ) ) ;
#21096=CARTESIAN_POINT ( 'NONE',  ( 2.774307903011629772, -278.5897569054384917, -206.9301572612380937 ) ) ;
#21098=CARTESIAN_POINT ( 'NONE',  ( -113.1714934331925377, -271.1395254068419263, -261.8434775121861549 ) ) ;
#21099=CARTESIAN_POINT ( 'NONE',  ( -61.83177852398269181, -276.7274862005567684, -339.2925720075747904 ) ) ;
#21100=CARTESIAN_POINT ( 'NONE',  ( 26.82886369925037684, -294.5797277384135668, -234.0237491028881038 ) ) ;
#21101=CARTESIAN_POINT ( 'NONE',  ( 27.37158344524206299, -294.9602609106559044, -304.7565312643018842 ) ) ;
#21102=CARTESIAN_POINT ( 'NONE',  ( -11.20980534635519810, -296.0339181902334076, -342.3229789612057061 ) ) ;
#21103=CARTESIAN_POINT ( 'NONE',  ( -107.6033856567162559, -296.1236479623738092, -290.1675702442213378 ) ) ;
#21104=CARTESIAN_POINT ( 'NONE',  ( -9.971109543656687890, -290.6950696756996422, -340.2441247845581529 ) ) ;
#21105=CARTESIAN_POINT ( 'NONE',  ( -105.7831740440014840, -284.2627908078724204, -305.7586700857913797 ) ) ;
#21106=CARTESIAN_POINT ( 'NONE',  ( -35.52919970570834352, -272.2142258109196291, -194.6050780441710231 ) ) ;
#21107=CARTESIAN_POINT ( 'NONE',  ( -30.88173815167097302, -285.9649563307573317, -193.6192828684417009 ) ) ;
#21108=CARTESIAN_POINT ( 'NONE',  ( -29.51647577905713504, -278.9325948321531428, -344.6466729639312234 ) ) ;
#21109=CARTESIAN_POINT ( 'NONE',  ( -5.686123378546612095, -285.5376497310342643, -204.3069002407272592 ) ) ;
#21110=CARTESIAN_POINT ( 'NONE',  ( -100.6276949432456860, -288.0092793917290805, -310.7045135057646235 ) ) ;
#21111=CARTESIAN_POINT ( 'NONE',  ( 122.2132510144744231, 146.9671518294229884, -260.0597590233358574 ) ) ;
#21112=CARTESIAN_POINT ( 'NONE',  ( 31.03440590732131099, -286.7148616216642836, -244.4753765253276754 ) ) ;
#21113=CARTESIAN_POINT ( 'NONE',  ( 19.61700487003165350, -283.1950339229233009, -321.9027351537781669 ) ) ;
#21114=CARTESIAN_POINT ( 'NONE',  ( -74.55430958609520076, -290.6282217033115671, -203.2191645515357266 ) ) ;
#21115=CARTESIAN_POINT ( 'NONE',  ( -48.02696793397387154, -281.5186604497420717, -194.8607274821272028 ) ) ;
#21116=CARTESIAN_POINT ( 'NONE',  ( -106.9772587562155195, -280.2764112352208485, -238.5445908078931438 ) ) ;
#21117=CARTESIAN_POINT ( 'NONE',  ( 2.705758260382665537, -280.4388651034481086, -209.2660366015047657 ) ) ;
#21118=CARTESIAN_POINT ( 'NONE',  ( -13.45184927674018738, -276.3625292210851399, -199.2676887956133953 ) ) ;
#21119=CARTESIAN_POINT ( 'NONE',  ( 8.906156743853365754, -294.4371410363464179, -331.9251962648914969 ) ) ;
#21120=CARTESIAN_POINT ( 'NONE',  ( -74.38258807489297908, -287.5673298601061560, -335.1818703558597008 ) ) ;
#21121=CARTESIAN_POINT ( 'NONE',  ( -27.96792527687896168, -293.7692496346715529, -194.6867571202456304 ) ) ;
#21122=CARTESIAN_POINT ( 'NONE',  ( -97.44465230440238201, -294.8896874827739794, -312.3356485179066908 ) ) ;
#21124=CARTESIAN_POINT ( 'NONE',  ( -10.43285348184764949, -284.6185987577881633, -339.8220185831044660 ) ) ;
#21125=CARTESIAN_POINT ( 'NONE',  ( -103.7360461296461551, -296.6301310111882685, -239.8440627133898886 ) ) ;
#21126=CARTESIAN_POINT ( 'NONE',  ( -13.97377717797410490, -293.4279248445182020, -197.2613249583244510 ) ) ;
#21127=CARTESIAN_POINT ( 'NONE',  ( 31.45334110770835068, -282.5341158614627375, -295.2319777552705773 ) ) ;
#21128=CARTESIAN_POINT ( 'NONE',  ( -63.46572195458924170, -272.7786107733008407, -198.1783243518403310 ) ) ;
#21129=CARTESIAN_POINT ( 'NONE',  ( -23.32236650191881111, -289.5289617630800194, -346.0244937158390712 ) ) ;
#21130=CARTESIAN_POINT ( 'NONE',  ( -0.9892477441648872549, -280.7145429992540926, -336.8499056821429463 ) ) ;
#21131=CARTESIAN_POINT ( 'NONE',  ( -112.9050191481909735, -291.0701167630201098, -255.5979045358685084 ) ) ;
#21132=CARTESIAN_POINT ( 'NONE',  ( 35.14571657019750006, -288.0016543015505022, -279.1737173247350938 ) ) ;
#21135=CARTESIAN_POINT ( 'NONE',  ( 202.4139397029900636, 292.0436245958289874, -68.22449661283333455 ) ) ;
#21136=CARTESIAN_POINT ( 'NONE',  ( -20.19161114001082069, -271.7666405000205714, -195.3683826091709363 ) ) ;
#21137=CARTESIAN_POINT ( 'NONE',  ( -76.90059059506310746, -278.7049333687505737, -208.7564712338032109 ) ) ;
#21139=CARTESIAN_POINT ( 'NONE',  ( -69.86510219893355611, -278.5337602417895937, -204.6474865008337076 ) ) ;
#21140=CARTESIAN_POINT ( 'NONE',  ( 2.410716822162965567, -274.2363688864952564, -204.4407900243765255 ) ) ;
#21141=CARTESIAN_POINT ( 'NONE',  ( 198.5597165885725133, 282.1031016261414948, -110.8136125372897993 ) ) ;
#21142=CARTESIAN_POINT ( 'NONE',  ( -56.39206956557844563, -278.3861985372600998, -196.3086388897377219 ) ) ;
#21143=CARTESIAN_POINT ( 'NONE',  ( -95.58387239043544525, -281.9268742885003007, -317.0686768613675213 ) ) ;
#21144=CARTESIAN_POINT ( 'NONE',  ( -86.81966061962245362, -299.1354330460225128, -212.6210731168986001 ) ) ;
#21145=CARTESIAN_POINT ( 'NONE',  ( 24.89700902263355431, -293.5162968812755366, -231.9985016091159480 ) ) ;
#21146=EDGE_LOOP ( 'NONE', ( #91677, #71969, #5321, #30801 ) ) ;
#21147=CARTESIAN_POINT ( 'NONE',  ( -103.9965963978455363, -289.6520629994708429, -239.4035941822990878 ) ) ;
#21148=CARTESIAN_POINT ( 'NONE',  ( 33.61628151908885798, -275.8246180384253989, -240.5878761696732226 ) ) ;
#21149=CARTESIAN_POINT ( 'NONE',  ( -55.29571555057212606, -297.9814996829738902, -199.5510982856281714 ) ) ;
#21154=CARTESIAN_POINT ( 'NONE',  ( -71.09618173569496946, -280.6754041129343022, -205.2711597043160054 ) ) ;
#21155=CARTESIAN_POINT ( 'NONE',  ( -38.18149286942044540, -281.8018979483874205, -194.3790887557871656 ) ) ;
#21157=CARTESIAN_POINT ( 'NONE',  ( -78.51878970601758567, -282.6805531654070478, -330.9239427311221675 ) ) ;
#21158=CARTESIAN_POINT ( 'NONE',  ( -41.13764488955257548, -281.8642833332503415, -196.2230286819362561 ) ) ;
#21159=CARTESIAN_POINT ( 'NONE',  ( 35.38826112719358008, -274.1912504007178768, -282.5458535948769168 ) ) ;
#21162=CARTESIAN_POINT ( 'NONE',  ( -22.95907811108590835, -277.6756135734006534, -345.8956448764176912 ) ) ;
#21165=CARTESIAN_POINT ( 'NONE',  ( 144.2857639756989272, -299.5541904835127980, -188.7068768330456123 ) ) ;
#21166=CARTESIAN_POINT ( 'NONE',  ( -67.20580790827278861, -285.4216638236208041, -339.5459564341089731 ) ) ;
#21167=CARTESIAN_POINT ( 'NONE',  ( 32.49790794043295250, -293.0375026586251010, -292.1563209385726054 ) ) ;
#21168=CARTESIAN_POINT ( 'NONE',  ( 27.35454246723739757, -287.4478698461635418, -312.0250026353834869 ) ) ;
#21169=CARTESIAN_POINT ( 'NONE',  ( -98.93814621192655068, -283.3538802424283745, -229.3263541432489205 ) ) ;
#21170=CARTESIAN_POINT ( 'NONE',  ( -69.01220709553993515, -284.2020079797344465, -203.9216675777556418 ) ) ;
#21171=CARTESIAN_POINT ( 'NONE',  ( -50.95960474744624946, -287.4682508542301775, -343.1632709709842857 ) ) ;
#21172=CARTESIAN_POINT ( 'NONE',  ( 20.50333807851700030, -283.3905603016838768, -315.5394541738708085 ) ) ;
#21173=CARTESIAN_POINT ( 'NONE',  ( -43.84331899308399727, -271.9699448504277939, -195.5915290422074122 ) ) ;
#21174=CARTESIAN_POINT ( 'NONE',  ( -66.86014849885927447, -284.0716050805226018, -200.1108395333039596 ) ) ;
#21175=CARTESIAN_POINT ( 'NONE',  ( -111.7925888053599408, -298.6686313517778331, -261.3020990961549046 ) ) ;
#21176=CARTESIAN_POINT ( 'NONE',  ( -70.24028501929326751, -283.6194677641286717, -202.7762709860772645 ) ) ;
#21177=CARTESIAN_POINT ( 'NONE',  ( -105.7383238995555814, -279.8435822688368830, -244.0405856772781306 ) ) ;
#21178=CARTESIAN_POINT ( 'NONE',  ( 30.05516742116387618, -289.9917707600530434, -303.7605733105853005 ) ) ;
#21181=CARTESIAN_POINT ( 'NONE',  ( 16.55193879744521013, -296.2138652272377044, -323.3958293713237140 ) ) ;
#21182=CARTESIAN_POINT ( 'NONE',  ( -112.3505877992131872, -276.5846707956379191, -267.8156500431153404 ) ) ;
#21183=CARTESIAN_POINT ( 'NONE',  ( -111.4743014381466963, -290.0035679183544062, -250.0994313474726880 ) ) ;
#21184=CARTESIAN_POINT ( 'NONE',  ( 29.10607921092357131, -292.3832851757165372, -302.5901628751475414 ) ) ;
#21185=CARTESIAN_POINT ( 'NONE',  ( -54.59240484389143688, -278.5107660067846496, -198.8686899550340854 ) ) ;
#21186=CARTESIAN_POINT ( 'NONE',  ( -66.02852212518352815, -295.8122873910523936, -201.8926454901307181 ) ) ;
#21187=CARTESIAN_POINT ( 'NONE',  ( -107.0442816173390241, -292.1746714847028557, -247.0631864953041372 ) ) ;
#21188=CARTESIAN_POINT ( 'NONE',  ( -106.6662871844225293, -275.4805209788416960, -237.0123917617630696 ) ) ;
#21189=CARTESIAN_POINT ( 'NONE',  ( 10.74623573116364916, -292.8814245578822693, -329.6766284268210256 ) ) ;
#21190=CARTESIAN_POINT ( 'NONE',  ( -93.00181338863293945, -291.4680984658751299, -318.8976727400695381 ) ) ;
#21191=CARTESIAN_POINT ( 'NONE',  ( 3.614486301459465700, -290.8344452406145706, -206.2943258002021309 ) ) ;
#21192=CARTESIAN_POINT ( 'NONE',  ( -34.53751184212538305, -290.4416423302682801, -343.9468823945292115 ) ) ;
#21194=CARTESIAN_POINT ( 'NONE',  ( -0.9021591587043433780, -289.3582565351172207, -333.8604446192612727 ) ) ;
#21196=CARTESIAN_POINT ( 'NONE',  ( -93.29222475175984641, -291.0392984489857326, -322.7591251942047279 ) ) ;
#21197=CARTESIAN_POINT ( 'NONE',  ( 36.08073246584901739, -279.3549051956842959, -253.3469468220091585 ) ) ;
#21198=CARTESIAN_POINT ( 'NONE',  ( -99.71160790639525828, -291.0745972829884636, -232.4270356327176614 ) ) ;
#21199=CARTESIAN_POINT ( 'NONE',  ( -79.90262721556769066, -279.8271021939681873, -206.1542720985193853 ) ) ;
#21200=CARTESIAN_POINT ( 'NONE',  ( 38.77447446082106808, -281.0707796424130152, -258.5230041031413180 ) ) ;
#21201=CARTESIAN_POINT ( 'NONE',  ( 37.55141082777899442, -285.4893312303795483, -265.4812786776086568 ) ) ;
#21202=CARTESIAN_POINT ( 'NONE',  ( -112.1436901920290268, -274.5519900738175920, -270.3865807095265268 ) ) ;
#21203=CARTESIAN_POINT ( 'NONE',  ( 34.84581001808292910, -279.9170585126622655, -287.7306951100896413 ) ) ;
#21205=CARTESIAN_POINT ( 'NONE',  ( -21.38401343115940278, -284.2566516355674366, -197.0784264318440933 ) ) ;
#21207=CARTESIAN_POINT ( 'NONE',  ( -113.5406919127116367, -276.9808909827281127, -274.4134509030984646 ) ) ;
#21208=CARTESIAN_POINT ( 'NONE',  ( 22.75826059940336066, -285.8322306536472297, -222.7010461313469989 ) ) ;
#21209=CARTESIAN_POINT ( 'NONE',  ( -37.83609679892234823, -298.9870633562416629, -197.1274916838459603 ) ) ;
#21211=CARTESIAN_POINT ( 'NONE',  ( -77.70960297263444261, -293.1002333730833698, -208.5802727794157931 ) ) ;
#21212=CARTESIAN_POINT ( 'NONE',  ( 36.70967539353675591, -276.7398320786147110, -251.5196722312257975 ) ) ;
#21213=CARTESIAN_POINT ( 'NONE',  ( -110.1897712811958598, -278.1434978350496294, -276.0763131487547639 ) ) ;
#21214=CARTESIAN_POINT ( 'NONE',  ( -14.97268084463497928, -296.7627049932192449, -342.0022565749762293 ) ) ;
#21215=CARTESIAN_POINT ( 'NONE',  ( -81.93211057851669921, -291.6294689600409811, -207.5861603931744526 ) ) ;
#21216=CARTESIAN_POINT ( 'NONE',  ( 19.07021333941937158, -278.9373534073271230, -220.0722790313181463 ) ) ;
#21217=CARTESIAN_POINT ( 'NONE',  ( -8.509249530970711461, -292.2526113399259771, -198.9630101849645030 ) ) ;
#21219=CARTESIAN_POINT ( 'NONE',  ( -108.6538487480726189, -289.8308538928027929, -253.6335571990357494 ) ) ;
#21220=CARTESIAN_POINT ( 'NONE',  ( -32.17635856413464523, -292.9868597423189840, -345.1959494806206408 ) ) ;
#21223=CARTESIAN_POINT ( 'NONE',  ( -1.220801655145375086, -292.0528605345135134, -206.8386057230477491 ) ) ;
#21226=CARTESIAN_POINT ( 'NONE',  ( 7.399455738971487229, -279.9094976428775681, -326.5171145203363494 ) ) ;
#21227=CARTESIAN_POINT ( 'NONE',  ( -109.2214567527080789, -295.2673111947250959, -297.4577819398419365 ) ) ;
#21228=CARTESIAN_POINT ( 'NONE',  ( -78.87785338044611194, -284.9147102337576030, -334.6109914841913451 ) ) ;
#21229=CARTESIAN_POINT ( 'NONE',  ( 33.99645877079259293, -287.1811639150399174, -254.8734748611770158 ) ) ;
#21230=CARTESIAN_POINT ( 'NONE',  ( -7.206584965477648375, -278.1696225689579478, -337.6112673372305153 ) ) ;
#21231=CARTESIAN_POINT ( 'NONE',  ( -34.25792316641321378, -293.0332903130373552, -344.9421955060753930 ) ) ;
#21232=CARTESIAN_POINT ( 'NONE',  ( -50.63146142528317029, -296.9843619659567935, -343.1715310827281655 ) ) ;
#21233=CARTESIAN_POINT ( 'NONE',  ( 21.14407994712002647, -274.9669138486726752, -314.7068509780767727 ) ) ;
#21236=CARTESIAN_POINT ( 'NONE',  ( -100.7308411919326971, -296.7959069380451638, -226.6623200645531142 ) ) ;
#21237=CARTESIAN_POINT ( 'NONE',  ( 17.08011511308455255, -290.1892874970391745, -321.2261365017562866 ) ) ;
#21238=CARTESIAN_POINT ( 'NONE',  ( 201.7538767631425003, 295.5538150823438173, -54.00000000004517631 ) ) ;
#21239=CARTESIAN_POINT ( 'NONE',  ( -23.44333400179391091, -299.3019944946597661, -193.6677463287124681 ) ) ;
#21240=CARTESIAN_POINT ( 'NONE',  ( 34.38578408321180291, -288.3902805497862687, -284.5347500568023520 ) ) ;
#21242=CARTESIAN_POINT ( 'NONE',  ( -45.23721179709964701, -279.0133500514301659, -193.9507026689990710 ) ) ;
#21243=CARTESIAN_POINT ( 'NONE',  ( 15.41478929567783318, -294.9810067277581425, -326.3081072673980429 ) ) ;
#21244=CARTESIAN_POINT ( 'NONE',  ( -43.11223418036092170, -287.2638671257919327, -345.9058492181630982 ) ) ;
#21245=CARTESIAN_POINT ( 'NONE',  ( -81.85601405369061467, -295.9733098157785207, -333.2292469481070611 ) ) ;
#21246=CARTESIAN_POINT ( 'NONE',  ( 35.22843514771243889, -293.9981606856766234, -278.9088006615419886 ) ) ;
#21250=CARTESIAN_POINT ( 'NONE',  ( -0.07190842257235939561, -288.0588134374509650, -203.7603954838894822 ) ) ;
#21251=CARTESIAN_POINT ( 'NONE',  ( -99.90806341382575795, -287.4094976428775112, -320.2154176792147382 ) ) ;
#21252=CARTESIAN_POINT ( 'NONE',  ( -33.91150779519067981, -279.4428342949065041, -193.5395938674784873 ) ) ;
#21253=CARTESIAN_POINT ( 'NONE',  ( -2.751879263566934242, -284.5939880970526019, -336.7348976013009860 ) ) ;
#21254=CARTESIAN_POINT ( 'NONE',  ( -113.2322969655488407, -283.2390573494901673, -261.4603537522617671 ) ) ;
#21255=CARTESIAN_POINT ( 'NONE',  ( -34.54798004935471312, -287.0967566587318629, -344.7992406314769482 ) ) ;
#21256=CARTESIAN_POINT ( 'NONE',  ( 18.01713818169475800, -278.1295158048703229, -322.0883303720370918 ) ) ;
#21257=CARTESIAN_POINT ( 'NONE',  ( -46.18554796405813789, -274.2701507500599405, -197.8775071302462720 ) ) ;
#21259=CARTESIAN_POINT ( 'NONE',  ( -101.8569219400553720, -278.0868628637650772, -304.5193696145124704 ) ) ;
#21260=CARTESIAN_POINT ( 'NONE',  ( -46.46096050094721619, -279.2820928344401636, -197.7790429055923198 ) ) ;
#21261=CARTESIAN_POINT ( 'NONE',  ( 22.50845317958115643, -275.9866561000245611, -222.3877001586689914 ) ) ;
#21262=CARTESIAN_POINT ( 'NONE',  ( -112.0112268252158430, -277.5620727571622979, -253.2593489650623724 ) ) ;
#21263=CARTESIAN_POINT ( 'NONE',  ( -113.6755508159304071, -270.8536776300014708, -283.8132029559086504 ) ) ;
#21264=CARTESIAN_POINT ( 'NONE',  ( -64.82706478045440690, -274.6430830346805010, -198.6714911177868714 ) ) ;
#21265=CARTESIAN_POINT ( 'NONE',  ( -91.23291200094298858, -298.7292094129201701, -216.1915363432169102 ) ) ;
#21266=CARTESIAN_POINT ( 'NONE',  ( -37.37352853689063892, -282.5519495502701943, -195.3611179825600175 ) ) ;
#21269=CARTESIAN_POINT ( 'NONE',  ( -62.68257507134601525, -286.7942446521547595, -201.5169626913884997 ) ) ;
#21270=CARTESIAN_POINT ( 'NONE',  ( -68.11124426436150259, -287.4138033428002359, -200.8688085861446950 ) ) ;
#21271=CARTESIAN_POINT ( 'NONE',  ( -39.97003480951236298, -288.4345010232981963, -343.4654341373205284 ) ) ;
#21272=CARTESIAN_POINT ( 'NONE',  ( -113.8433405749718474, -283.9573355507500310, -278.5480534333684091 ) ) ;
#21273=CARTESIAN_POINT ( 'NONE',  ( -14.03713971575828978, -278.7592937563051692, -200.2832497034550272 ) ) ;
#21274=CARTESIAN_POINT ( 'NONE',  ( -44.16103738394220102, -287.8254229133307263, -196.4397941343143827 ) ) ;
#21275=CARTESIAN_POINT ( 'NONE',  ( 32.00047629107431391, -280.3629305433468630, -295.4592362771664398 ) ) ;
#21276=CARTESIAN_POINT ( 'NONE',  ( -13.61041993946012418, -278.0528513790765714, -339.9708546693551625 ) ) ;
#21277=CARTESIAN_POINT ( 'NONE',  ( 19.04234870993378337, -275.3865622127032680, -223.8979338634113390 ) ) ;
#21278=CARTESIAN_POINT ( 'NONE',  ( -38.92741896036859117, -287.8665624559097864, -346.9476325643174732 ) ) ;
#21279=CARTESIAN_POINT ( 'NONE',  ( 26.59321056689514506, -282.9171417432854128, -312.9813715582304212 ) ) ;
#21280=CARTESIAN_POINT ( 'NONE',  ( -99.29841921454772091, -285.6520062994288196, -224.6566554609867126 ) ) ;
#21281=CARTESIAN_POINT ( 'NONE',  ( -16.92374966210020304, -280.4899794279351113, -200.2746905999659646 ) ) ;
#21285=CARTESIAN_POINT ( 'NONE',  ( -64.97409137456668304, -291.2695786855250617, -340.9626785477648241 ) ) ;
#21286=CARTESIAN_POINT ( 'NONE',  ( -84.87149853817895462, -288.3765489830022375, -330.3805074032717357 ) ) ;
#21287=CARTESIAN_POINT ( 'NONE',  ( -64.64541401129325493, -272.7454639000781071, -202.3923483293288541 ) ) ;
#21288=CARTESIAN_POINT ( 'NONE',  ( 6.549008573836617053, -293.8216718229184607, -333.5680453066373730 ) ) ;
#21290=CARTESIAN_POINT ( 'NONE',  ( -109.0293439096645756, -288.8088678295441127, -287.4371094214757250 ) ) ;
#21291=CARTESIAN_POINT ( 'NONE',  ( 13.61685543193546089, -291.0177947290402471, -216.6843108199037147 ) ) ;
#21292=CARTESIAN_POINT ( 'NONE',  ( 33.46905300474775657, -289.0132223566969856, -289.8622422578415581 ) ) ;
#21293=CARTESIAN_POINT ( 'NONE',  ( -114.2704648735229114, -287.0519495502703080, -270.3937649182068981 ) ) ;
#21294=CARTESIAN_POINT ( 'NONE',  ( 18.16176755763629203, -290.2562433903181613, -320.8219611049982518 ) ) ;
#21295=CARTESIAN_POINT ( 'NONE',  ( -111.3332659755394900, -288.3814470593611077, -283.6731627468009833 ) ) ;
#21297=CARTESIAN_POINT ( 'NONE',  ( -23.52876731164776203, -294.2287434121942624, -196.5919547122190920 ) ) ;
#21298=CARTESIAN_POINT ( 'NONE',  ( -105.4282743961954196, -285.1320848982025495, -297.4736639907682729 ) ) ;
#21299=CARTESIAN_POINT ( 'NONE',  ( -39.19270091967422331, -294.0291617513930191, -195.2045166616555321 ) ) ;
#21302=CARTESIAN_POINT ( 'NONE',  ( -102.8132364824645748, -275.0283573855661530, -232.9483691663406546 ) ) ;
#21303=CARTESIAN_POINT ( 'NONE',  ( 12.01811760469106005, -281.5416795939549957, -324.3630635026745495 ) ) ;
#21304=CARTESIAN_POINT ( 'NONE',  ( -93.17039472124659483, -281.8542081279704803, -320.4619591663890787 ) ) ;
#21305=CARTESIAN_POINT ( 'NONE',  ( -97.28789784910350136, -295.1037172037462142, -318.4507722160524281 ) ) ;
#21306=CARTESIAN_POINT ( 'NONE',  ( 28.77644220285192134, -273.3467712171160997, -237.0990485095763631 ) ) ;
#21307=CARTESIAN_POINT ( 'NONE',  ( -109.8951831907875487, -276.4158429125819225, -287.0702036927465883 ) ) ;
#21308=CARTESIAN_POINT ( 'NONE',  ( -52.75474825975436488, -299.1658246299951429, -198.4501195967229989 ) ) ;
#21309=CARTESIAN_POINT ( 'NONE',  ( -0.4469370417777366322, -295.9770761929294736, -334.0915021885120382 ) ) ;
#21312=CARTESIAN_POINT ( 'NONE',  ( 6.167159403133554818, -295.2476099321969514, -329.2424614016791224 ) ) ;
#21314=CARTESIAN_POINT ( 'NONE',  ( 27.30083539783106161, -285.0550641877488260, -231.5338303023210926 ) ) ;
#21315=CARTESIAN_POINT ( 'NONE',  ( -93.08239456204718465, -295.8820380417219553, -317.5183125269336415 ) ) ;
#21316=CARTESIAN_POINT ( 'NONE',  ( -78.52246274269717219, -285.5139667304173940, -205.2984959136742589 ) ) ;
#21317=CARTESIAN_POINT ( 'NONE',  ( 37.80337648723936894, -287.4285663488244040, -287.1234291388756219 ) ) ;
#21318=CARTESIAN_POINT ( 'NONE',  ( -92.46862867832687982, -297.8161907965251203, -321.7554842977831413 ) ) ;
#21319=CARTESIAN_POINT ( 'NONE',  ( -19.61375188303495065, -290.2803447588852919, -197.6043799376736558 ) ) ;
#21320=CARTESIAN_POINT ( 'NONE',  ( -72.42394825665984115, -278.7970112352028877, -201.9842667297878620 ) ) ;
#21321=CARTESIAN_POINT ( 'NONE',  ( -110.4542110544635705, -294.2666405000204577, -253.6410175316879361 ) ) ;
#21323=CARTESIAN_POINT ( 'NONE',  ( -25.06035422671212487, -285.0070351367819512, -197.9472632055166343 ) ) ;
#21325=CARTESIAN_POINT ( 'NONE',  ( -76.94589455299046676, -287.5825399559333846, -334.0518428317784583 ) ) ;
#21326=CARTESIAN_POINT ( 'NONE',  ( -106.5632221731606819, -298.4915293816200688, -244.6241271892120608 ) ) ;
#21327=CARTESIAN_POINT ( 'NONE',  ( 23.26874848992852662, -282.3517029414020953, -223.8104058276473154 ) ) ;
#21328=CARTESIAN_POINT ( 'NONE',  ( -112.1390381335946813, -294.6892204006201723, -261.2087942729142469 ) ) ;
#21329=CARTESIAN_POINT ( 'NONE',  ( 35.42901951167450392, -281.6364471782130181, -276.7511404148033307 ) ) ;
#21330=CARTESIAN_POINT ( 'NONE',  ( -112.6009524058867868, -296.9231587029738648, -254.0193672505807854 ) ) ;
#21331=CARTESIAN_POINT ( 'NONE',  ( -95.08627725284839016, -274.6159676476437426, -224.7438106114496179 ) ) ;
#21332=CARTESIAN_POINT ( 'NONE',  ( 0.8159999791476266751, -284.6367183790358126, -205.1287033498456083 ) ) ;
#21334=CARTESIAN_POINT ( 'NONE',  ( -35.41365353264124138, -282.0764801100624481, -195.3731042840245777 ) ) ;
#21335=CARTESIAN_POINT ( 'NONE',  ( -69.34958648091600253, -296.6790175942991823, -204.4907630406402461 ) ) ;
#21337=CARTESIAN_POINT ( 'NONE',  ( 83.14890176555634582, -297.1582149144751384, -195.3611179825600175 ) ) ;
#21338=CARTESIAN_POINT ( 'NONE',  ( -85.91338271712612595, -285.7089061417845528, -327.0412595688014790 ) ) ;
#21340=CARTESIAN_POINT ( 'NONE',  ( -85.28047601435909542, -288.9094976428777386, -210.1954327657594206 ) ) ;
#21341=CARTESIAN_POINT ( 'NONE',  ( 23.38413236604104384, -275.3795324871163643, -317.4625141535940429 ) ) ;
#21342=CARTESIAN_POINT ( 'NONE',  ( 20.99508032478530950, -292.7692238509437175, -226.4769516930897169 ) ) ;
#21343=CARTESIAN_POINT ( 'NONE',  ( 21.87466388457362854, -282.4627592899136062, -226.4749804589744429 ) ) ;
#21344=CARTESIAN_POINT ( 'NONE',  ( 26.07329512816975736, -277.6656207090827593, -308.1100092324665525 ) ) ;
#21345=CARTESIAN_POINT ( 'NONE',  ( 25.28458159991488685, -283.7319798563980839, -313.7936272354587004 ) ) ;
#21346=CARTESIAN_POINT ( 'NONE',  ( 22.44580575025058877, -279.7555805469957591, -227.7866579592388803 ) ) ;
#21347=CARTESIAN_POINT ( 'NONE',  ( -84.23801284099724285, -279.6968515522974599, -328.9577323644639364 ) ) ;
#21348=CARTESIAN_POINT ( 'NONE',  ( -99.56830686352940063, -273.3217635584348386, -224.9202005216477858 ) ) ;
#21349=CARTESIAN_POINT ( 'NONE',  ( -2.727012337184489432, -276.4405986332532734, -339.1567771311206911 ) ) ;
#21350=CARTESIAN_POINT ( 'NONE',  ( 6.938773765591287557, -296.3647515999579127, -330.2631006016060837 ) ) ;
#21353=CARTESIAN_POINT ( 'NONE',  ( 8.145370589423139407, -292.5770245399876899, -330.9518093089620265 ) ) ;
#21354=CARTESIAN_POINT ( 'NONE',  ( -35.38239740990338333, -273.5850209208139745, -197.3133396504947257 ) ) ;
#21356=CARTESIAN_POINT ( 'NONE',  ( 31.61187946678717253, -295.4962844463024680, -303.1663340991964333 ) ) ;
#21357=CARTESIAN_POINT ( 'NONE',  ( 24.48485388998581769, -294.1536275444740340, -225.1340692437146629 ) ) ;
#21358=CARTESIAN_POINT ( 'NONE',  ( 15.39294038702397494, -290.3048975160289729, -323.4561847501590819 ) ) ;
#21360=CARTESIAN_POINT ( 'NONE',  ( -112.1838994929950530, -276.5846707936894973, -267.8212503199704315 ) ) ;
#21361=CARTESIAN_POINT ( 'NONE',  ( -41.92121508043608458, -279.0304350080685367, -344.6729685723889816 ) ) ;
#21362=CARTESIAN_POINT ( 'NONE',  ( 35.05384187436523291, -291.4071984988084978, -252.9803134857809823 ) ) ;
#21363=CARTESIAN_POINT ( 'NONE',  ( 19.19098021615143068, -282.7173128192280842, -219.8999530194980139 ) ) ;
#21364=CARTESIAN_POINT ( 'NONE',  ( -105.8489335441694976, -283.8194352437740804, -244.2654278646709542 ) ) ;
#21366=CARTESIAN_POINT ( 'NONE',  ( -21.38772728848908500, -282.5087210543082961, -341.6701325559633915 ) ) ;
#21367=CARTESIAN_POINT ( 'NONE',  ( -72.37790729830854275, -280.6792107811446044, -202.1266101619298468 ) ) ;
#21368=CARTESIAN_POINT ( 'NONE',  ( -101.0972352662010252, -282.7842157071579550, -312.9209014827710575 ) ) ;
#21369=CARTESIAN_POINT ( 'NONE',  ( -105.9706143199053940, -279.9384947163266020, -235.8494913762532406 ) ) ;
#21370=CARTESIAN_POINT ( 'NONE',  ( -86.63244065416141382, -279.2425828732394280, -328.6808230668561350 ) ) ;
#21371=CARTESIAN_POINT ( 'NONE',  ( 27.33386217378599881, -295.6233781216987495, -239.1787733560258573 ) ) ;
#21374=CARTESIAN_POINT ( 'NONE',  ( -58.49254416103472920, -299.7788533544078859, -198.4052812288414316 ) ) ;
#21375=CARTESIAN_POINT ( 'NONE',  ( -104.8467963803897050, -276.9946683709684976, -238.3820821732341244 ) ) ;
#21376=CARTESIAN_POINT ( 'NONE',  ( -85.88315453333730431, -293.1509498526403945, -211.8316718680007966 ) ) ;
#21377=CARTESIAN_POINT ( 'NONE',  ( -3.103347651892360393, -293.9357373727264644, -334.9492584431066007 ) ) ;
#21378=CARTESIAN_POINT ( 'NONE',  ( -98.11485749106958565, -289.4292078704581854, -317.5432146682532561 ) ) ;
#21380=CARTESIAN_POINT ( 'NONE',  ( -4.770303547612166462, -293.2062836189126074, -339.4964591033963757 ) ) ;
#21381=CARTESIAN_POINT ( 'NONE',  ( -90.22201717344397309, -283.6891000058087116, -218.8085621058053505 ) ) ;
#21382=CARTESIAN_POINT ( 'NONE',  ( -3.087005893952967206, -294.3701665050123211, -204.5015597877963671 ) ) ;
#21383=CARTESIAN_POINT ( 'NONE',  ( 16.49407922800606840, -285.3147434412307462, -220.0193685667901491 ) ) ;
#21384=CARTESIAN_POINT ( 'NONE',  ( 33.80511217668076540, -283.1094891608026387, -288.8334127336015626 ) ) ;
#21385=CARTESIAN_POINT ( 'NONE',  ( -65.34996963061553288, -290.3505630567544813, -341.8900559315690657 ) ) ;
#21386=CARTESIAN_POINT ( 'NONE',  ( -11.72744321366486275, -280.8870908776754050, -201.8832194128696074 ) ) ;
#21387=CARTESIAN_POINT ( 'NONE',  ( 39.31428347453377370, -292.3466305283561155, -270.3255398957106195 ) ) ;
#21388=CARTESIAN_POINT ( 'NONE',  ( 21.37225936225295442, -289.0241304790955610, -319.9275358679049077 ) ) ;
#21389=CARTESIAN_POINT ( 'NONE',  ( -106.4554723598231334, -290.6086741439372645, -304.2877217913605818 ) ) ;
#21390=CARTESIAN_POINT ( 'NONE',  ( -100.9923601050083590, -285.2091427361062301, -234.5140787532585023 ) ) ;
#21392=CARTESIAN_POINT ( 'NONE',  ( 31.12414629204448602, -295.8365236657332389, -302.9293497766255427 ) ) ;
#21393=CARTESIAN_POINT ( 'NONE',  ( -113.8159819983055598, -295.2825359508860856, -266.7417986598027255 ) ) ;
#21394=CARTESIAN_POINT ( 'NONE',  ( -95.46705930252035444, -276.9861388340378880, -314.9127853999037256 ) ) ;
#21395=CARTESIAN_POINT ( 'NONE',  ( -113.0066083995344997, -272.2378554502179213, -256.1359044117549502 ) ) ;
#21396=CARTESIAN_POINT ( 'NONE',  ( -6.492130255045490017, -293.1193271474610356, -337.2865376154775845 ) ) ;
#21397=CARTESIAN_POINT ( 'NONE',  ( 36.38553290198070300, -277.2204548159018600, -263.3021088964512160 ) ) ;
#21398=CARTESIAN_POINT ( 'NONE',  ( -92.01650251236651457, -271.4006516052635902, -220.1274546884554013 ) ) ;
#21399=CARTESIAN_POINT ( 'NONE',  ( 24.77142996404363018, -295.2955861353386240, -309.5601941021214429 ) ) ;
#21400=CARTESIAN_POINT ( 'NONE',  ( -67.40947196203978820, -296.5357082085511138, -337.2340997557380433 ) ) ;
#21402=CARTESIAN_POINT ( 'NONE',  ( -88.34516788969136769, -295.3398691568279446, -215.0758281356166322 ) ) ;
#21403=CARTESIAN_POINT ( 'NONE',  ( -30.50418177803270936, -298.7870618871939996, -193.4623166349295502 ) ) ;
#21404=CARTESIAN_POINT ( 'NONE',  ( 27.54148833797076890, -286.5976912020086615, -305.1905063281713524 ) ) ;
#21406=CARTESIAN_POINT ( 'NONE',  ( -107.9494543833702807, -291.2351393495428056, -289.9889099853360790 ) ) ;
#21407=CARTESIAN_POINT ( 'NONE',  ( -95.98485595537673021, -273.7166013571282406, -220.5361407569864696 ) ) ;
#21408=CARTESIAN_POINT ( 'NONE',  ( -110.3955101695432433, -296.9068586695804584, -268.7366596028214758 ) ) ;
#21409=CARTESIAN_POINT ( 'NONE',  ( -112.7387722004195609, -280.5161268319159831, -271.6069157584847744 ) ) ;
#21410=CARTESIAN_POINT ( 'NONE',  ( 14.83732007160970845, -279.4536524782851075, -214.3364869631018053 ) ) ;
#21411=ORIENTED_EDGE ( 'NONE', *, *, #60434, .T. ) ;
#21412=CARTESIAN_POINT ( 'NONE',  ( -31.65211809747334826, -282.3307269029556892, -347.0616648443773897 ) ) ;
#21413=CARTESIAN_POINT ( 'NONE',  ( 38.39316699270343491, -274.7329365952886633, -256.9613168756970936 ) ) ;
#21414=CARTESIAN_POINT ( 'NONE',  ( 37.35723688023576727, -280.1422294028776605, -285.4113414819611307 ) ) ;
#21415=CARTESIAN_POINT ( 'NONE',  ( -14.75381922397232870, -278.3438646986959384, -198.6140320828808683 ) ) ;
#21417=CARTESIAN_POINT ( 'NONE',  ( -70.67636136704722105, -296.2878382342544796, -204.8486874361631749 ) ) ;
#21418=CARTESIAN_POINT ( 'NONE',  ( -32.17872436761616939, -276.1174149492999845, -195.5262770011973714 ) ) ;
#21420=CARTESIAN_POINT ( 'NONE',  ( -34.98601919685224004, -290.1016805967838081, -195.0298743235898371 ) ) ;
#21422=CARTESIAN_POINT ( 'NONE',  ( -99.20459208274296259, -291.1618868005963350, -224.4916465671718129 ) ) ;
#21423=CARTESIAN_POINT ( 'NONE',  ( -54.92994582530294423, -275.8266867040787247, -197.2811478351008248 ) ) ;
#21424=CARTESIAN_POINT ( 'NONE',  ( -99.48648187488048222, -271.1211597239678213, -228.2800997367835407 ) ) ;
#21425=CARTESIAN_POINT ( 'NONE',  ( -103.8954707845855125, -284.2508101692046694, -231.8528003569259681 ) ) ;
#21428=CARTESIAN_POINT ( 'NONE',  ( -111.6166571419884406, -282.4138117147431899, -281.1228031932268436 ) ) ;
#21430=CARTESIAN_POINT ( 'NONE',  ( 33.69636507485748211, -292.1046990867142199, -251.9024127719551984 ) ) ;
#21431=CARTESIAN_POINT ( 'NONE',  ( -30.39245392472972185, -284.2804099009798051, -196.4002347469137248 ) ) ;
#21434=CARTESIAN_POINT ( 'NONE',  ( 21.24041447881314681, -292.1961249494211188, -317.2125168805756630 ) ) ;
#21435=CARTESIAN_POINT ( 'NONE',  ( -113.5175605608882989, -282.9652824982334209, -275.6502607883592191 ) ) ;
#21436=CARTESIAN_POINT ( 'NONE',  ( -59.99839998567912147, -281.3538685891093678, -200.0710908577658529 ) ) ;
#21437=CARTESIAN_POINT ( 'NONE',  ( -109.6077781263779514, -286.0794158120244788, -244.9520115678777756 ) ) ;
#21438=CARTESIAN_POINT ( 'NONE',  ( -2.830081744852734005, -278.7417935764178196, -202.6492986790875932 ) ) ;
#21439=CARTESIAN_POINT ( 'NONE',  ( 34.56739659606086690, -287.3825311905106332, -257.5029209381216901 ) ) ;
#21440=CARTESIAN_POINT ( 'NONE',  ( -54.07037762220355859, -278.6963128482075831, -342.0762630842294811 ) ) ;
#21441=CARTESIAN_POINT ( 'NONE',  ( -110.4410605348046772, -279.3153154961788687, -273.3752902739163346 ) ) ;
#21443=CARTESIAN_POINT ( 'NONE',  ( -8.007199267271198906, -288.4142652374155205, -200.8946324920737538 ) ) ;
#21445=CARTESIAN_POINT ( 'NONE',  ( -20.50779345604741621, -298.0907843225825786, -193.3615769139673546 ) ) ;
#21446=CARTESIAN_POINT ( 'NONE',  ( 35.90289766715125808, -289.7185447161817251, -284.8174295038053856 ) ) ;
#21448=CARTESIAN_POINT ( 'NONE',  ( -115.3288506153726871, -280.8376638359844151, -288.1938231032136741 ) ) ;
#21450=CARTESIAN_POINT ( 'NONE',  ( -66.79327125728174508, -271.6670034999890504, -201.2045319864713235 ) ) ;
#21451=CARTESIAN_POINT ( 'NONE',  ( 36.98554331911887516, -291.7391773340946770, -253.5126277257724894 ) ) ;
#21452=CARTESIAN_POINT ( 'NONE',  ( -41.38009691863028650, -287.5205441174657039, -196.7659005114314823 ) ) ;
#21453=CARTESIAN_POINT ( 'NONE',  ( 27.33360214868353566, -282.8269776044406285, -234.3739079380453347 ) ) ;
#21454=CARTESIAN_POINT ( 'NONE',  ( 37.44304227898425097, -288.7790141760688698, -254.6182756471966968 ) ) ;
#21455=CARTESIAN_POINT ( 'NONE',  ( 31.25274891271851629, -289.3068945009376876, -304.3642733043050725 ) ) ;
#21456=CARTESIAN_POINT ( 'NONE',  ( -112.3915647492318328, -286.5447593930720700, -270.9497396867755583 ) ) ;
#21457=CARTESIAN_POINT ( 'NONE',  ( -108.6556342216229467, -278.3500133887044399, -299.4011387916142439 ) ) ;
#21459=CARTESIAN_POINT ( 'NONE',  ( -33.53235727059151827, -293.0844331167886594, -345.8379114322244732 ) ) ;
#21460=CARTESIAN_POINT ( 'NONE',  ( -11.50735574411731399, -280.2127311159050578, -197.7683400477946520 ) ) ;
#21461=CARTESIAN_POINT ( 'NONE',  ( -111.5777819524823684, -274.4482009412615753, -267.6148025881067269 ) ) ;
#21462=CARTESIAN_POINT ( 'NONE',  ( -4.771743288812468897, -285.1233781216987495, -337.9199732462171255 ) ) ;
#21463=CARTESIAN_POINT ( 'NONE',  ( -91.43179795749590255, -271.5349147600256856, -216.9922569333990623 ) ) ;
#21465=CARTESIAN_POINT ( 'NONE',  ( -62.32410252672553241, -279.2260164632038482, -201.6501033849325495 ) ) ;
#21466=CARTESIAN_POINT ( 'NONE',  ( 38.52877522146756917, -276.6243737987749682, -259.7932568615818241 ) ) ;
#21467=CARTESIAN_POINT ( 'NONE',  ( -33.79447898179370924, -299.5226837574093111, -196.7710040749456653 ) ) ;
#21468=CARTESIAN_POINT ( 'NONE',  ( -113.3680671762393075, -283.4729469363727503, -281.3582739984130399 ) ) ;
#21469=CARTESIAN_POINT ( 'NONE',  ( -100.5890149847064237, -292.8344549044419409, -231.9195886729019662 ) ) ;
#21470=CARTESIAN_POINT ( 'NONE',  ( -43.99344572504309525, -275.5696530276545673, -194.3992417064939673 ) ) ;
#21471=CARTESIAN_POINT ( 'NONE',  ( 30.33659482775287586, -300.0868488860655816, -193.7446608145621951 ) ) ;
#21472=CARTESIAN_POINT ( 'NONE',  ( -17.71576201847185317, -296.7985928871418082, -342.5750430728895708 ) ) ;
#21473=CARTESIAN_POINT ( 'NONE',  ( -5.269760757205497193, -280.6290538853249359, -337.9874824674561751 ) ) ;
#21474=CARTESIAN_POINT ( 'NONE',  ( -67.00337498109597334, -291.3405669656972918, -199.3264128274505538 ) ) ;
#21475=CARTESIAN_POINT ( 'NONE',  ( -46.35289299348226422, -271.9573501466052790, -196.2622299715482654 ) ) ;
#21476=CARTESIAN_POINT ( 'NONE',  ( -46.43050066141889687, -287.5387672241343466, -194.7050929796331786 ) ) ;
#21477=CARTESIAN_POINT ( 'NONE',  ( -84.01530829273427514, -290.3132741877302578, -213.8297074788579550 ) ) ;
#21479=CARTESIAN_POINT ( 'NONE',  ( -95.02550210999098113, -288.4443523301134178, -320.4728459797386790 ) ) ;
#21480=CARTESIAN_POINT ( 'NONE',  ( -90.77176297467201493, -290.9345193009630748, -220.5699900472900481 ) ) ;
#21482=CARTESIAN_POINT ( 'NONE',  ( -57.68721897056022385, -286.8752286527841306, -196.3630864068943254 ) ) ;
#21483=CARTESIAN_POINT ( 'NONE',  ( -68.04244926072802002, -277.7999790617918734, -336.6285594747408254 ) ) ;
#21484=CARTESIAN_POINT ( 'NONE',  ( 34.17955452696386942, -292.1187557242975004, -242.5339279771212091 ) ) ;
#21485=CARTESIAN_POINT ( 'NONE',  ( -97.08794490109738717, -284.5531681626406453, -318.7935735132654713 ) ) ;
#21486=CARTESIAN_POINT ( 'NONE',  ( -112.3400891012334171, -285.1024653158666524, -253.0121715273484426 ) ) ;
#21487=CARTESIAN_POINT ( 'NONE',  ( -49.14950696976872280, -280.2308000225204978, -198.3009820939238921 ) ) ;
#21488=CARTESIAN_POINT ( 'NONE',  ( 185.6829310669746462, 263.5356091243360765, -153.4021477105963243 ) ) ;
#21490=CARTESIAN_POINT ( 'NONE',  ( 63.70159209483512797, 48.22975029174962458, -318.1369363225185793 ) ) ;
#21491=CARTESIAN_POINT ( 'NONE',  ( -56.80084188927647659, -168.8182197709074046, -361.0463781639207923 ) ) ;
#21493=CARTESIAN_POINT ( 'NONE',  ( -90.30646721055705939, -272.4757563819280790, -219.8716600230470419 ) ) ;
#21494=CARTESIAN_POINT ( 'NONE',  ( -34.01294384033642615, -273.0153285925379691, -197.1276184363042603 ) ) ;
#21495=CARTESIAN_POINT ( 'NONE',  ( -101.5803473206244973, -295.5015107232558194, -312.8004037482381818 ) ) ;
#21496=CARTESIAN_POINT ( 'NONE',  ( -101.3485003382535723, -255.0465241227205979, -324.4801213465552792 ) ) ;
#21497=CARTESIAN_POINT ( 'NONE',  ( -7.864996635055389262, -273.1150887667228062, -199.7044361416253082 ) ) ;
#21498=CARTESIAN_POINT ( 'NONE',  ( -69.81895627968575013, -299.4802318397225349, -203.6071419447495430 ) ) ;
#21499=CARTESIAN_POINT ( 'NONE',  ( 32.78922225733731466, -289.1586181643885993, -292.5055419561649614 ) ) ;
#21501=CARTESIAN_POINT ( 'NONE',  ( -97.17052517212012219, -298.1399411993618287, -222.2640088382701151 ) ) ;
#21503=CARTESIAN_POINT ( 'NONE',  ( 24.99996933245994057, -287.5200207195633766, -232.2625000227118335 ) ) ;
#21504=CARTESIAN_POINT ( 'NONE',  ( -78.66338643976456524, -272.4297658651656207, -205.7545335686023122 ) ) ;
#21505=CARTESIAN_POINT ( 'NONE',  ( 22.16807974827314709, -295.0090052377701113, -318.9898516642721802 ) ) ;
#21506=CARTESIAN_POINT ( 'NONE',  ( -37.68240824331939365, -295.5486197407395821, -347.3118934514236571 ) ) ;
#21507=CARTESIAN_POINT ( 'NONE',  ( 33.77590485901108508, -293.9367662397261824, -286.8869646159539002 ) ) ;
#21509=CARTESIAN_POINT ( 'NONE',  ( -68.27729901727558115, -275.5691788448407920, -201.4100406849607339 ) ) ;
#21512=CARTESIAN_POINT ( 'NONE',  ( -112.4257248369146254, -277.8496532722548409, -287.1514764392074426 ) ) ;
#21513=CARTESIAN_POINT ( 'NONE',  ( 35.41777855516782125, -273.7899004003899677, -257.9369021103371438 ) ) ;
#21514=CARTESIAN_POINT ( 'NONE',  ( -37.16397723159514044, -299.2595114767989912, -196.9611406590407512 ) ) ;
#21515=CARTESIAN_POINT ( 'NONE',  ( 34.12550975376370133, -276.7044817918813351, -286.4133811976718675 ) ) ;
#21516=CARTESIAN_POINT ( 'NONE',  ( -64.55834345259904694, -275.4618401520278326, -199.4018682670943576 ) ) ;
#21517=CARTESIAN_POINT ( 'NONE',  ( -17.80906853067696360, -274.8215773215832201, -343.1408067894699343 ) ) ;
#21518=CARTESIAN_POINT ( 'NONE',  ( -106.9638098869072138, -296.9064867921208020, -292.8106757444147092 ) ) ;
#21519=CARTESIAN_POINT ( 'NONE',  ( 8.581832049218400371, -292.9838561365360761, -327.9279346713149721 ) ) ;
#21521=CARTESIAN_POINT ( 'NONE',  ( -109.5506113879550014, -279.3821693467757541, -243.6479029370459841 ) ) ;
#21522=CARTESIAN_POINT ( 'NONE',  ( -37.80762893467147734, -277.2247927442888340, -343.3720839985188036 ) ) ;
#21523=CARTESIAN_POINT ( 'NONE',  ( 38.30054579420336580, -286.0915161927486565, -258.8042906515589721 ) ) ;
#21524=CARTESIAN_POINT ( 'NONE',  ( -85.20778782822631570, -297.7116797421144270, -328.3168430817167973 ) ) ;
#21525=CARTESIAN_POINT ( 'NONE',  ( 82.65856464842170226, -298.7952694379614513, -197.7495342522536816 ) ) ;
#21526=CARTESIAN_POINT ( 'NONE',  ( 17.94084266078888490, -287.4314508133875279, -318.3581640327193440 ) ) ;
#21527=CARTESIAN_POINT ( 'NONE',  ( -93.51008306804587278, -276.1152376563603070, -318.5595284676081178 ) ) ;
#21528=CARTESIAN_POINT ( 'NONE',  ( -110.7451143679794399, -277.1952637989844561, -265.1348675249990947 ) ) ;
#21529=CARTESIAN_POINT ( 'NONE',  ( -78.37709724978498116, -285.6040486583280540, -333.2005340795712982 ) ) ;
#21530=CARTESIAN_POINT ( 'NONE',  ( -91.24911084563214558, -279.0449886155982426, -320.2458855676034091 ) ) ;
#21532=CARTESIAN_POINT ( 'NONE',  ( 38.13461029507453759, -273.8196222189280320, -259.8841441783870323 ) ) ;
#21533=CARTESIAN_POINT ( 'NONE',  ( 33.93128985157731137, -275.9888409818506716, -254.0554553733323075 ) ) ;
#21534=CARTESIAN_POINT ( 'NONE',  ( 15.90596991672398097, -282.8041539367392829, -217.2342810461550187 ) ) ;
#21536=CARTESIAN_POINT ( 'NONE',  ( -18.06760574957008103, -290.7257349571830787, -343.4215277896019529 ) ) ;
#21537=CARTESIAN_POINT ( 'NONE',  ( 35.80217473764341918, -291.3383509234745929, -253.7219851101134509 ) ) ;
#21539=CARTESIAN_POINT ( 'NONE',  ( -90.54211130835216181, -271.9634975908120964, -219.6380786202479953 ) ) ;
#21540=CARTESIAN_POINT ( 'NONE',  ( 23.61552052922447942, -291.1108102924919763, -227.9702939864256450 ) ) ;
#21541=CARTESIAN_POINT ( 'NONE',  ( 206.6943913402143096, 294.1769577359763161, -83.83314285352493300 ) ) ;
#21543=CARTESIAN_POINT ( 'NONE',  ( -100.1212885157644052, -288.4540303298966819, -313.7365837998821689 ) ) ;
#21544=CARTESIAN_POINT ( 'NONE',  ( -83.27691636625509375, -285.2933055698237013, -328.1882256796054094 ) ) ;
#21545=CARTESIAN_POINT ( 'NONE',  ( -35.15464261151896608, -284.3190904410691928, -194.3929583529316290 ) ) ;
#21546=CARTESIAN_POINT ( 'NONE',  ( -36.16605991260344410, -284.4624008067302725, -343.9409575375638610 ) ) ;
#21547=CARTESIAN_POINT ( 'NONE',  ( -109.5822001631679967, -285.5083508857517813, -258.7096648739631632 ) ) ;
#21548=CARTESIAN_POINT ( 'NONE',  ( -112.0392307135613095, -292.6638894053500053, -260.0440852111001391 ) ) ;
#21550=CARTESIAN_POINT ( 'NONE',  ( 13.94722594299829410, -275.0816345629415309, -212.8861406575224748 ) ) ;
#21552=CARTESIAN_POINT ( 'NONE',  ( -90.60121189453791146, -287.8790595574993745, -324.0326797218828574 ) ) ;
#21553=CARTESIAN_POINT ( 'NONE',  ( -59.66501024252430341, -277.3335391814662785, -344.0541965282037040 ) ) ;
#21554=CARTESIAN_POINT ( 'NONE',  ( 32.12532965656419037, -295.8909301638625493, -297.8189301995707865 ) ) ;
#21556=CARTESIAN_POINT ( 'NONE',  ( -20.25526795762937127, -294.7662352645559167, -195.3538533559490702 ) ) ;
#21557=CARTESIAN_POINT ( 'NONE',  ( -103.9252033361590435, -283.6557015111425812, -239.1297574213755297 ) ) ;
#21558=CARTESIAN_POINT ( 'NONE',  ( -78.78388096887881886, -277.4940363649671440, -207.7884632752493133 ) ) ;
#21559=CARTESIAN_POINT ( 'NONE',  ( -104.9852800969474771, -271.4930346039406004, -234.9333220023199260 ) ) ;
#21560=CARTESIAN_POINT ( 'NONE',  ( 35.12264531535633694, -274.7738262835058549, -260.7272554324752036 ) ) ;
#21562=CARTESIAN_POINT ( 'NONE',  ( 0.2461993104067672911, -294.0827168792916382, -206.9745455221475936 ) ) ;
#21563=CARTESIAN_POINT ( 'NONE',  ( -5.951614167666416044, -293.4164558207309597, -204.1803000874634506 ) ) ;
#21565=CARTESIAN_POINT ( 'NONE',  ( 25.32043023167499385, -295.4517254781991369, -314.2788136781078947 ) ) ;
#21566=CARTESIAN_POINT ( 'NONE',  ( -93.08376905849242178, -295.7153849568382498, -317.5166878978336626 ) ) ;
#21567=CARTESIAN_POINT ( 'NONE',  ( -105.8649150796414631, -292.1513018780649418, -300.9781217295776514 ) ) ;
#21568=CARTESIAN_POINT ( 'NONE',  ( -70.46819411277715517, -283.6434715493737713, -339.8855456207680277 ) ) ;
#21569=CARTESIAN_POINT ( 'NONE',  ( -68.31704371975510526, -271.7892202014795657, -201.2033839585289456 ) ) ;
#21570=CARTESIAN_POINT ( 'NONE',  ( -43.66415077770040654, -285.8078088627343618, -193.5678651683101350 ) ) ;
#21571=CARTESIAN_POINT ( 'NONE',  ( -110.6540620784711706, -280.3500343965315551, -284.4693485422583308 ) ) ;
#21573=CARTESIAN_POINT ( 'NONE',  ( -46.74323606647199369, -284.9887471177253246, -197.6808494438146511 ) ) ;
#21574=CARTESIAN_POINT ( 'NONE',  ( -108.8820235597720796, -288.2595304863650654, -293.0472499839460170 ) ) ;
#21575=CARTESIAN_POINT ( 'NONE',  ( 79.80194596570532894, 84.98805272827966917, -300.3302785054510196 ) ) ;
#21576=CARTESIAN_POINT ( 'NONE',  ( -57.40527084919665413, -285.2938994737045277, -200.0557638606933040 ) ) ;
#21577=CARTESIAN_POINT ( 'NONE',  ( 34.94784481344460403, -282.4341265075883030, -244.8605167064576165 ) ) ;
#21578=CARTESIAN_POINT ( 'NONE',  ( -23.36657542224108397, -287.9365528975321809, -345.8969585413705090 ) ) ;
#21579=CARTESIAN_POINT ( 'NONE',  ( -112.2751674014556187, -279.9765246838028361, -284.2680182883651128 ) ) ;
#21580=CARTESIAN_POINT ( 'NONE',  ( -110.1919046225565779, -279.5696502051916355, -293.9013367939087402 ) ) ;
#21581=CARTESIAN_POINT ( 'NONE',  ( -104.4412340725470330, -278.7717087096538080, -241.6095519570272927 ) ) ;
#21582=CARTESIAN_POINT ( 'NONE',  ( -51.90653774012873356, -275.8448939105290947, -197.0981018425740672 ) ) ;
#21583=CARTESIAN_POINT ( 'NONE',  ( 23.97522895132989618, -292.9312602574916582, -223.7643822824878441 ) ) ;
#21585=CARTESIAN_POINT ( 'NONE',  ( 2.161127084883642357, -286.5404046667965758, -333.6965223306931989 ) ) ;
#21586=CARTESIAN_POINT ( 'NONE',  ( -47.65549479289109769, -293.5233823838627814, -194.8090988526867307 ) ) ;
#21589=CARTESIAN_POINT ( 'NONE',  ( -102.8021862705189875, -295.9198773675413463, -237.2458457095668507 ) ) ;
#21590=CARTESIAN_POINT ( 'NONE',  ( -29.26457252396425801, -284.8693241671346641, -344.4131197844662324 ) ) ;
#21591=CARTESIAN_POINT ( 'NONE',  ( -72.13839101902910045, -295.1925262915897861, -334.5725704725780361 ) ) ;
#21592=CARTESIAN_POINT ( 'NONE',  ( 20.13785987141878664, -293.9413351344625198, -219.5712840788302742 ) ) ;
#21593=CARTESIAN_POINT ( 'NONE',  ( 18.03632735017891520, -281.5246799537732159, -222.6222371292827518 ) ) ;
#21594=CARTESIAN_POINT ( 'NONE',  ( 37.40854832670542862, -274.3910895064950637, -252.8333351820176063 ) ) ;
#21595=CARTESIAN_POINT ( 'NONE',  ( -108.7007811131989001, -290.8393973437330260, -299.0176067291662889 ) ) ;
#21596=CARTESIAN_POINT ( 'NONE',  ( -55.43060388946867079, -281.4220826753064557, -343.9348703573852504 ) ) ;
#21597=CARTESIAN_POINT ( 'NONE',  ( -114.0910319812618638, -290.8029316756999947, -276.9560068633767287 ) ) ;
#21598=CARTESIAN_POINT ( 'NONE',  ( -14.56343679039542671, -286.6888367987467063, -200.9305803135136159 ) ) ;
#21600=CARTESIAN_POINT ( 'NONE',  ( 201.2091503359040132, 294.9048254156658118, -54.00000000001405454 ) ) ;
#21601=CARTESIAN_POINT ( 'NONE',  ( 201.9872660792514125, 292.2036060437295646, -68.21650457366665421 ) ) ;
#21602=CARTESIAN_POINT ( 'NONE',  ( -102.0044027273109890, -277.2841595008096078, -304.5859133658730116 ) ) ;
#21603=CARTESIAN_POINT ( 'NONE',  ( -66.17868379056844219, -278.5859360690672020, -202.9482055685049033 ) ) ;
#21604=CARTESIAN_POINT ( 'NONE',  ( -44.03668832469244876, -273.6365553024820088, -193.6206584673421389 ) ) ;
#21605=CARTESIAN_POINT ( 'NONE',  ( 204.3872521652993157, 292.5237103994863332, -68.38542364661543616 ) ) ;
#21606=CARTESIAN_POINT ( 'NONE',  ( -104.2686865475563565, -277.6081331592102401, -233.4912823404381186 ) ) ;
#21607=CARTESIAN_POINT ( 'NONE',  ( -33.43479398991843965, -281.0228628273752634, -344.9164644161824071 ) ) ;
#21608=CARTESIAN_POINT ( 'NONE',  ( -107.9553395524242347, -298.6746570177957096, -242.1538334752297317 ) ) ;
#21609=CARTESIAN_POINT ( 'NONE',  ( -101.1804965051250917, -291.5311892881917970, -234.7241560361980817 ) ) ;
#21610=CARTESIAN_POINT ( 'NONE',  ( 20.73693582700091298, -286.8672207463941959, -315.4160909995291036 ) ) ;
#21611=CARTESIAN_POINT ( 'NONE',  ( 26.84090953594390427, -275.6458511372166527, -228.0065975243298908 ) ) ;
#21612=CARTESIAN_POINT ( 'NONE',  ( -91.12253635318792533, -273.2607672393718303, -220.9804657552562333 ) ) ;
#21617=CARTESIAN_POINT ( 'NONE',  ( -93.90046042582240204, -281.1640195211295463, -220.2570180196736089 ) ) ;
#21621=CARTESIAN_POINT ( 'NONE',  ( -24.83712607667366612, -281.2951122896281504, -198.1263500339461530 ) ) ;
#21622=CARTESIAN_POINT ( 'NONE',  ( 20.28280433913066361, -282.6345698065748024, -220.8096281756893973 ) ) ;
#21623=CARTESIAN_POINT ( 'NONE',  ( -65.41694875149451605, -282.4871414713202853, -338.0149038646231361 ) ) ;
#21624=CARTESIAN_POINT ( 'NONE',  ( -102.9374943536818563, -279.9469793518366600, -305.1182360674529264 ) ) ;
#21625=CARTESIAN_POINT ( 'NONE',  ( -91.62022936201221057, -271.7408906481244912, -220.4971930892697287 ) ) ;
#21632=CARTESIAN_POINT ( 'NONE',  ( -98.66835631091346670, -278.7369042413498619, -316.6774179278179986 ) ) ;
#21634=CARTESIAN_POINT ( 'NONE',  ( -48.42658574098470581, -275.7651966918988933, -346.0170591924380687 ) ) ;
#21637=CARTESIAN_POINT ( 'NONE',  ( -111.3869487363219264, -286.7142499958719668, -256.0995608770604122 ) ) ;
#21639=CARTESIAN_POINT ( 'NONE',  ( 31.95727912934837178, -292.4364572166456924, -246.7458711093032662 ) ) ;
#21640=CARTESIAN_POINT ( 'NONE',  ( 25.76329977371850433, -287.4832734677033841, -314.3964932657501663 ) ) ;
#21641=CARTESIAN_POINT ( 'NONE',  ( -105.5224159068926753, -283.1748125050613680, -241.4308018029734342 ) ) ;
#21642=CARTESIAN_POINT ( 'NONE',  ( -95.41091995294009109, -283.7589359383159717, -225.1373372570798495 ) ) ;
#21643=CARTESIAN_POINT ( 'NONE',  ( -7.834832642210999509, -286.9001114519323323, -338.2931316660093444 ) ) ;
#21644=CARTESIAN_POINT ( 'NONE',  ( -51.07723978435029011, -284.4365651535318307, -342.5133578590064758 ) ) ;
#21645=CARTESIAN_POINT ( 'NONE',  ( -57.55739002344556354, -271.7911514768463235, -198.0829970067160275 ) ) ;
#21646=CARTESIAN_POINT ( 'NONE',  ( -98.68793262238550312, -283.5598688821616520, -225.0738840330492394 ) ) ;
#21647=CARTESIAN_POINT ( 'NONE',  ( -63.54299156843381979, -297.3938025511578189, -340.6355299356363275 ) ) ;
#21648=CARTESIAN_POINT ( 'NONE',  ( -37.94163254081603753, -284.0444955546336132, -195.1968411470654132 ) ) ;
#21650=CARTESIAN_POINT ( 'NONE',  ( -71.06063647708360520, -280.5370070859619318, -205.3358944144751490 ) ) ;
#21651=CARTESIAN_POINT ( 'NONE',  ( -3.081797100774910980, -288.5037884121805405, -203.4416555286214816 ) ) ;
#21654=CARTESIAN_POINT ( 'NONE',  ( 36.38437959071472250, -295.6839235819234091, -286.9658801958458412 ) ) ;
#21656=CARTESIAN_POINT ( 'NONE',  ( -111.4726614747209226, -276.4058186460673596, -281.7453711091009154 ) ) ;
#21657=CARTESIAN_POINT ( 'NONE',  ( -103.6642287301438472, -289.2420868535085106, -309.2669111937612456 ) ) ;
#21658=CARTESIAN_POINT ( 'NONE',  ( -80.64042831410260703, -294.0503834968018282, -330.1244892959138610 ) ) ;
#21659=CARTESIAN_POINT ( 'NONE',  ( -24.77571488164446123, -278.9006523987242190, -197.9502107130680315 ) ) ;
#21660=CARTESIAN_POINT ( 'NONE',  ( -86.23798008150411931, -271.4478677781171427, -214.1634056662846035 ) ) ;
#21661=CARTESIAN_POINT ( 'NONE',  ( -19.97174117925349179, -293.5951458085277181, -198.8975187062117129 ) ) ;
#21662=CARTESIAN_POINT ( 'NONE',  ( -54.49178911615188525, -276.3376638359844719, -195.3683826091709363 ) ) ;
#21663=CARTESIAN_POINT ( 'NONE',  ( 8.474283869770276922, -292.9172637434522812, -331.3824532780968752 ) ) ;
#21664=CARTESIAN_POINT ( 'NONE',  ( -0.5753915663916416845, -290.1554236723253553, -334.4096276911703853 ) ) ;
#21665=CARTESIAN_POINT ( 'NONE',  ( -5.014621696398503303, -290.7117910480880028, -201.5938727460895734 ) ) ;
#21666=CARTESIAN_POINT ( 'NONE',  ( 26.21402754858381812, -289.4836882163552332, -307.5569713674225341 ) ) ;
#21668=CARTESIAN_POINT ( 'NONE',  ( -104.1911113380295717, -290.9541666594027447, -300.2142578689294510 ) ) ;
#21669=DIRECTION ( 'NONE',  ( 1.000000000000000000, 0.000000000000000000, 0.000000000000000000 ) ) ;
#21670=CARTESIAN_POINT ( 'NONE',  ( -23.36922114259783001, -290.0825351749548418, -345.7328052492806592 ) ) ;
#21671=CARTESIAN_POINT ( 'NONE',  ( 22.45777935031969363, -278.9470893438970052, -224.4877774330086595 ) ) ;
#21672=CARTESIAN_POINT ( 'NONE',  ( -110.3678007572729030, -290.5772078642548877, -268.4617592813915508 ) ) ;
#21673=CARTESIAN_POINT ( 'NONE',  ( -94.94878642804771118, -279.5774029742238440, -219.3006841850539956 ) ) ;
#21674=CARTESIAN_POINT ( 'NONE',  ( 37.52681219251520162, -281.4434688679618262, -288.3184521114259837 ) ) ;
#21675=CARTESIAN_POINT ( 'NONE',  ( 35.95588706133857215, -285.3479802348275598, -254.4719907163343748 ) ) ;
#21677=CARTESIAN_POINT ( 'NONE',  ( 34.96886250822412734, -279.4738751420048857, -253.5668327880892718 ) ) ;
#21678=CARTESIAN_POINT ( 'NONE',  ( -95.99983296993552528, -283.1944355236548745, -223.6254345568210908 ) ) ;
#21680=CARTESIAN_POINT ( 'NONE',  ( -90.56061837288628169, -277.7949446385939609, -215.6024258239367555 ) ) ;
#21681=CARTESIAN_POINT ( 'NONE',  ( -85.30882903859010469, -284.3271952661763180, -210.5226098715470471 ) ) ;
#21682=CARTESIAN_POINT ( 'NONE',  ( -93.90973673680072409, -274.0109500682585804, -223.9447701593392992 ) ) ;
#21684=CARTESIAN_POINT ( 'NONE',  ( -111.1049168002749070, -292.1052211301469583, -273.9681564387738604 ) ) ;
#21685=CARTESIAN_POINT ( 'NONE',  ( 34.16391560519255677, -276.6340024219124984, -243.4250230463540845 ) ) ;
#21686=CARTESIAN_POINT ( 'NONE',  ( 17.44828432164722543, -275.9081584519254875, -318.6515565660632774 ) ) ;
#21687=CARTESIAN_POINT ( 'NONE',  ( -58.96106121763084218, -297.3320423909741521, -342.1775776033581451 ) ) ;
#21688=CARTESIAN_POINT ( 'NONE',  ( -26.14246142706570453, -289.0800028626284757, -346.5423299511843993 ) ) ;
#21689=CARTESIAN_POINT ( 'NONE',  ( 23.08845653405152021, -280.2472594782648798, -315.7209059740592352 ) ) ;
#21690=CARTESIAN_POINT ( 'NONE',  ( 19.41709738036474064, -292.6775777614255958, -218.3280620478390972 ) ) ;
#21691=CARTESIAN_POINT ( 'NONE',  ( -70.31595892442398110, -290.6651600909797253, -204.9691711874021678 ) ) ;
#21693=CARTESIAN_POINT ( 'NONE',  ( -47.38951087331584944, -293.1796984727084237, -344.6850182177905708 ) ) ;
#21697=CARTESIAN_POINT ( 'NONE',  ( -55.02118321038742010, -291.3262505632821444, -199.4708907336494121 ) ) ;
#21699=CARTESIAN_POINT ( 'NONE',  ( -80.81485487069150508, -286.4195236320518347, -207.0284344941582049 ) ) ;
#21700=CARTESIAN_POINT ( 'NONE',  ( -53.28691492658257545, -271.3380690714491266, -200.3538533559491555 ) ) ;
#21701=CARTESIAN_POINT ( 'NONE',  ( -19.35408185640407197, -293.8850963931893148, -345.0433476254814309 ) ) ;
#21702=CARTESIAN_POINT ( 'NONE',  ( -67.67035877338909700, -284.7570530858516804, -340.5997878055861179 ) ) ;
#21703=CARTESIAN_POINT ( 'NONE',  ( -104.5967266486639460, -284.7680172284426021, -241.8452622724917660 ) ) ;
#21705=CARTESIAN_POINT ( 'NONE',  ( 16.11401278437593731, -277.7965801984698828, -321.0877826620890687 ) ) ;
#21706=CARTESIAN_POINT ( 'NONE',  ( 36.53923402363708561, -291.4348426970789774, -259.7096217587803721 ) ) ;
#21707=CARTESIAN_POINT ( 'NONE',  ( 35.71054697486245288, -295.1565824653816321, -258.3932275606181861 ) ) ;
#21709=CARTESIAN_POINT ( 'NONE',  ( -32.40912050689573931, -275.7836397569085420, -343.6424984516066843 ) ) ;
#21712=CARTESIAN_POINT ( 'NONE',  ( 26.49183720988387947, -293.7858838100850676, -313.3846441332607355 ) ) ;
#21713=CARTESIAN_POINT ( 'NONE',  ( 37.07056929121656452, -289.5168318378418917, -273.8024871024016988 ) ) ;
#21714=CARTESIAN_POINT ( 'NONE',  ( 201.6526253774845543, 295.4708909185295056, -54.00000000003612399 ) ) ;
#21715=AXIS2_PLACEMENT_3D ( 'NONE', #55900, #26059, #26546 ) ;
#21716=CARTESIAN_POINT ( 'NONE',  ( 53.12040451806458918, -300.2394943505627225, -193.6540424337711670 ) ) ;
#21717=CARTESIAN_POINT ( 'NONE',  ( -54.78869651922693862, -286.4734590947068114, -199.3193451868030763 ) ) ;
#21719=CARTESIAN_POINT ( 'NONE',  ( -56.48635047578894586, -278.8701409524386463, -195.9671829698715442 ) ) ;
#21720=CARTESIAN_POINT ( 'NONE',  ( -44.77749932147799683, -295.7952024755983871, -346.9521676764430254 ) ) ;
#21721=CARTESIAN_POINT ( 'NONE',  ( -38.91860484509828666, -287.2113282747291692, -346.1095097492282093 ) ) ;
#21722=CARTESIAN_POINT ( 'NONE',  ( -113.1823023974315277, -296.7166740914675529, -283.8511490800067349 ) ) ;
#21723=CARTESIAN_POINT ( 'NONE',  ( 14.88766405255949543, -293.1466135064929404, -219.2575238806394680 ) ) ;
#21728=CARTESIAN_POINT ( 'NONE',  ( -18.37326389616899647, -287.8122263031095827, -196.3950398920317753 ) ) ;
#21729=CARTESIAN_POINT ( 'NONE',  ( 36.57525178469694538, -291.4809262143062369, -305.9938812882205070 ) ) ;
#21731=CARTESIAN_POINT ( 'NONE',  ( -106.0807342157223729, -278.3460858061934005, -235.7714311475588715 ) ) ;
#21732=CARTESIAN_POINT ( 'NONE',  ( -31.98978832152237572, -284.9846209702211013, -345.0028319717018803 ) ) ;
#21733=CARTESIAN_POINT ( 'NONE',  ( -80.58964352083211224, -284.0533803937519224, -207.3034389648248066 ) ) ;
#21735=CARTESIAN_POINT ( 'NONE',  ( -15.45107799362714296, -286.8465849420167046, -341.5635195849741308 ) ) ;
#21736=CARTESIAN_POINT ( 'NONE',  ( -20.37922041317234090, -278.6970899088186684, -344.2565487930448285 ) ) ;
#21737=CARTESIAN_POINT ( 'NONE',  ( -66.84993899834188369, -298.1471030697205151, -203.5099194421589459 ) ) ;
#21739=CARTESIAN_POINT ( 'NONE',  ( 33.21898569042035376, -292.5075653531688999, -290.9594915361004723 ) ) ;
#21740=CARTESIAN_POINT ( 'NONE',  ( -85.10524184118780511, -277.7330176942925277, -325.6335496229921773 ) ) ;
#21741=CARTESIAN_POINT ( 'NONE',  ( -93.16267359623789446, -278.5708008655215622, -223.1411073630389126 ) ) ;
#21742=CARTESIAN_POINT ( 'NONE',  ( -21.43238691046070699, -275.3312447751002310, -195.3385463002959739 ) ) ;
#21743=CARTESIAN_POINT ( 'NONE',  ( -109.2282164417697032, -277.6850198581814197, -243.7441700496726185 ) ) ;
#21744=CARTESIAN_POINT ( 'NONE',  ( 199.7491719457015620, 292.1072351560490006, -82.63401296664939366 ) ) ;
#21745=CARTESIAN_POINT ( 'NONE',  ( -104.0793581943162422, -297.4900294610848164, -307.6806784570537729 ) ) ;
#21746=CARTESIAN_POINT ( 'NONE',  ( -37.30987171927208124, -279.5519495502701943, -345.3611179825600175 ) ) ;
#21747=CARTESIAN_POINT ( 'NONE',  ( 82.68081405346485724, -297.0478052522023518, -195.0828515018483529 ) ) ;
#21748=CARTESIAN_POINT ( 'NONE',  ( -11.92766018874138290, -287.4705866327009858, -201.5980999603520729 ) ) ;
#21750=CARTESIAN_POINT ( 'NONE',  ( -113.1427923795099844, -286.3884599297053910, -264.3510049481332658 ) ) ;
#21751=CARTESIAN_POINT ( 'NONE',  ( 17.89711178524258983, -287.5828457132016638, -318.3176477992096807 ) ) ;
#21752=CARTESIAN_POINT ( 'NONE',  ( -97.99977793551259708, -283.4269155914028033, -317.6910715030023198 ) ) ;
#21753=CARTESIAN_POINT ( 'NONE',  ( -41.07145826836466540, -278.4042980647125773, -196.6554240337372335 ) ) ;
#21754=CARTESIAN_POINT ( 'NONE',  ( -94.35577204744396340, -285.7491435983187102, -317.9033211951823432 ) ) ;
#21755=CARTESIAN_POINT ( 'NONE',  ( 33.98978738806516020, -280.2746516633096689, -288.9188051615073505 ) ) ;
#21757=CARTESIAN_POINT ( 'NONE',  ( -40.51037746368601233, -278.4079712347958093, -343.7984783205209851 ) ) ;
#21758=CARTESIAN_POINT ( 'NONE',  ( 20.07471269429220584, -276.6814959992061631, -315.5625027960275588 ) ) ;
#21759=CARTESIAN_POINT ( 'NONE',  ( 7.688634765473509880, -287.2478717357618621, -332.3964949390118022 ) ) ;
#21760=CARTESIAN_POINT ( 'NONE',  ( -52.87495473942416169, -284.0490481734789796, -345.6675826657482844 ) ) ;
#21761=CARTESIAN_POINT ( 'NONE',  ( 33.51170862437711406, -282.4280025500357851, -300.4858884375234993 ) ) ;
#21765=CARTESIAN_POINT ( 'NONE',  ( -54.20329078882887330, -291.1267332211077132, -344.2796373406740713 ) ) ;
#21766=CARTESIAN_POINT ( 'NONE',  ( -97.06800996909851165, -289.8815949450092262, -222.5482934687692875 ) ) ;
#21767=CARTESIAN_POINT ( 'NONE',  ( -81.20237167259689670, -272.4984748850349092, -211.6489631753028391 ) ) ;
#21768=CARTESIAN_POINT ( 'NONE',  ( 37.32496265445777084, -292.6703791436969482, -251.9708418573292192 ) ) ;
#21769=CARTESIAN_POINT ( 'NONE',  ( -89.16223791121014131, -288.2774164101108454, -322.7571065274370881 ) ) ;
#21770=CARTESIAN_POINT ( 'NONE',  ( 7.305105622832725132, -290.9101547363768532, -211.3303061364287032 ) ) ;
#21771=CARTESIAN_POINT ( 'NONE',  ( 36.02762337789592095, -288.8018686036191411, -273.7630125538476022 ) ) ;
#21772=CARTESIAN_POINT ( 'NONE',  ( -110.4542110544635705, -292.8376638359844719, -287.0812184334320705 ) ) ;
#21774=CARTESIAN_POINT ( 'NONE',  ( -43.00518548740925695, -291.1238205171648588, -345.1469828421396642 ) ) ;
#21775=CARTESIAN_POINT ( 'NONE',  ( -109.7821149103507707, -288.2945442640377678, -290.4213955173162844 ) ) ;
#21776=CARTESIAN_POINT ( 'NONE',  ( -97.03941445755313566, -293.1737498562713427, -224.9401512154376803 ) ) ;
#21777=CARTESIAN_POINT ( 'NONE',  ( -90.90540367049743509, -284.7774704727244170, -320.3044669999755456 ) ) ;
#21778=CARTESIAN_POINT ( 'NONE',  ( -5.406741242633555267, -294.4714841033494963, -202.3156417773798523 ) ) ;
#21782=CARTESIAN_POINT ( 'NONE',  ( -65.63358930329401630, -275.6639188389321475, -200.5047410037102509 ) ) ;
#21783=CARTESIAN_POINT ( 'NONE',  ( -40.25099234621683308, -282.2868198995290072, -343.4647276480588403 ) ) ;
#21784=CARTESIAN_POINT ( 'NONE',  ( -64.81096724150229704, -281.4107401070241963, -340.1496558204850089 ) ) ;
#21785=CARTESIAN_POINT ( 'NONE',  ( -114.2049636948820819, -295.7230768984458678, -272.4551688669206442 ) ) ;
#21786=CARTESIAN_POINT ( 'NONE',  ( -59.76155105279463697, -271.9976995216208024, -199.7714892471298640 ) ) ;
#21787=CARTESIAN_POINT ( 'NONE',  ( -71.12780261895926515, -275.5815619626100670, -336.6922078231229420 ) ) ;
#21788=CARTESIAN_POINT ( 'NONE',  ( -88.48084421931424970, -298.6323826213073858, -217.5071803188237993 ) ) ;
#21790=CARTESIAN_POINT ( 'NONE',  ( 6.427858286978637814, -295.8699494810848591, -329.5820562702344318 ) ) ;
#21792=CARTESIAN_POINT ( 'NONE',  ( -0.6681704988668493161, -295.3547369127751949, -333.7249769427886008 ) ) ;
#21794=CARTESIAN_POINT ( 'NONE',  ( 32.34812088404733998, -285.1984743357985508, -241.5587551745245207 ) ) ;
#21795=CARTESIAN_POINT ( 'NONE',  ( -109.7362330339659025, -296.6809605365436937, -260.5967397307236979 ) ) ;
#21797=CARTESIAN_POINT ( 'NONE',  ( -97.17239457006462544, -283.9018604790301197, -318.8512924680750871 ) ) ;
#21798=CARTESIAN_POINT ( 'NONE',  ( 27.12237205103609128, -286.6659975600267103, -228.2882325385497779 ) ) ;
#21799=CARTESIAN_POINT ( 'NONE',  ( 22.47419734123972646, -290.9360399087347560, -225.3934980815385813 ) ) ;
#21800=CARTESIAN_POINT ( 'NONE',  ( -73.68023496432654440, -278.7795507255493135, -202.6433952533539582 ) ) ;
#21801=CARTESIAN_POINT ( 'NONE',  ( -37.30987171927208834, -277.5523547857346784, -195.3611179825600175 ) ) ;
#21804=CARTESIAN_POINT ( 'NONE',  ( 33.46087754133158398, -286.6034603034618158, -289.8918952704985941 ) ) ;
#21805=CARTESIAN_POINT ( 'NONE',  ( -113.8784774835396689, -289.5335016852888543, -265.5016714038294481 ) ) ;
#21808=CARTESIAN_POINT ( 'NONE',  ( -104.6580641169477133, -297.7477578156853610, -300.7340600901302992 ) ) ;
#21809=CARTESIAN_POINT ( 'NONE',  ( -96.14021537502127046, -293.9268482520018893, -317.5105341253381539 ) ) ;
#21810=CARTESIAN_POINT ( 'NONE',  ( -1.952115106104068909, -280.2014284063606055, -206.4888645481774176 ) ) ;
#21811=CARTESIAN_POINT ( 'NONE',  ( -68.22423139129976732, -295.6133665174211274, -340.8967066403378681 ) ) ;
#21812=CARTESIAN_POINT ( 'NONE',  ( -110.2254087330158399, -280.3244697979502007, -288.1056715706646969 ) ) ;
#21813=CARTESIAN_POINT ( 'NONE',  ( -106.0223267440893551, -295.9505583568613361, -244.7909038657860776 ) ) ;
#21816=CARTESIAN_POINT ( 'NONE',  ( -36.14237516623786206, -285.0169309673198654, -344.9962868110795853 ) ) ;
#21818=CARTESIAN_POINT ( 'NONE',  ( -95.99890600148557951, -287.4094976428776249, -317.0979686699210447 ) ) ;
#21819=CARTESIAN_POINT ( 'NONE',  ( -2.806864703871376321, -275.8045490108797821, -339.0161603780088058 ) ) ;
#21820=CARTESIAN_POINT ( 'NONE',  ( -17.43055719457050401, -292.1495172258112234, -200.0764356445261569 ) ) ;
#21821=CARTESIAN_POINT ( 'NONE',  ( 29.59441305995499150, -282.6588529956806042, -239.4125356282316375 ) ) ;
#21822=CARTESIAN_POINT ( 'NONE',  ( -51.73724255811971062, -275.4651912250458849, -197.9263790437122168 ) ) ;
#21823=CARTESIAN_POINT ( 'NONE',  ( -34.48831178038967238, -284.6169690265235204, -346.5076779307435686 ) ) ;
#21824=CARTESIAN_POINT ( 'NONE',  ( 21.31805035291759864, -280.9634454126324385, -314.4972323636638976 ) ) ;
#21825=CARTESIAN_POINT ( 'NONE',  ( -106.0948902248394461, -280.1586023692168510, -300.4577895527651208 ) ) ;
#21826=CARTESIAN_POINT ( 'NONE',  ( 53.58753502002358715, -299.1611516537437296, -193.3610657143116782 ) ) ;
#21827=CARTESIAN_POINT ( 'NONE',  ( 39.38032164253318967, -275.4672258268549285, -276.8980423297837206 ) ) ;
#21828=CARTESIAN_POINT ( 'NONE',  ( 33.72876223152904629, -295.7600498889233904, -292.5039176749680223 ) ) ;
#21831=CARTESIAN_POINT ( 'NONE',  ( 12.56411675703698272, -292.5052596951728674, -327.4369296289947897 ) ) ;
#21832=CARTESIAN_POINT ( 'NONE',  ( -38.07669348961997002, -273.5503480781993062, -197.3032763320682932 ) ) ;
#21834=CARTESIAN_POINT ( 'NONE',  ( -53.26371836535142990, -293.3718100777188056, -195.6800550602520730 ) ) ;
#21835=CARTESIAN_POINT ( 'NONE',  ( 31.98288692825981272, -278.4805209788417528, -303.7098442033569654 ) ) ;
#21836=CARTESIAN_POINT ( 'NONE',  ( -27.91326286185599059, -293.3742606311471377, -194.2872419503543426 ) ) ;
#21837=CARTESIAN_POINT ( 'NONE',  ( -56.51124884301842854, -291.2998115444024734, -342.7514043404716517 ) ) ;
#21838=CARTESIAN_POINT ( 'NONE',  ( -108.8765098679053551, -276.2660599907086976, -292.5075319989022660 ) ) ;
#21839=CARTESIAN_POINT ( 'NONE',  ( -79.42635005625847100, -279.5450601268025252, -331.8257965372164335 ) ) ;
#21840=CARTESIAN_POINT ( 'NONE',  ( 33.17283793648693546, -291.3193158478521241, -246.3464828689928936 ) ) ;
#21841=CARTESIAN_POINT ( 'NONE',  ( 35.30128606378762157, -283.6890844606402311, -292.0662504952661038 ) ) ;
#21843=CARTESIAN_POINT ( 'NONE',  ( 11.92782979010978650, -282.0111553900312629, -324.2554674854873724 ) ) ;
#21844=CARTESIAN_POINT ( 'NONE',  ( -61.96146498611592079, -280.8192414426507071, -197.6734361564319897 ) ) ;
#21846=CARTESIAN_POINT ( 'NONE',  ( -95.04578693486982388, -282.6621991725297676, -320.7421370779891276 ) ) ;
#21847=CARTESIAN_POINT ( 'NONE',  ( -113.9964095188055921, -279.4418686648850780, -274.4691273028197429 ) ) ;
#21850=CARTESIAN_POINT ( 'NONE',  ( 12.26866339178549836, -277.8961259548783005, -328.3397311290792118 ) ) ;
#21851=CARTESIAN_POINT ( 'NONE',  ( -67.74223827176244583, -282.1233781216987495, -207.3071070584150277 ) ) ;
#21854=CARTESIAN_POINT ( 'NONE',  ( -73.84190424486551763, -299.5675580659681145, -204.8421455432032587 ) ) ;
#21855=CIRCLE ( 'NONE', #17101, 2.186979415864515275 ) ;
#21856=CARTESIAN_POINT ( 'NONE',  ( -67.48958005552772477, -275.4697008299434060, -338.6469301346039060 ) ) ;
#21857=CARTESIAN_POINT ( 'NONE',  ( -42.01434047100565294, -293.7541517698392113, -194.5182511676785566 ) ) ;
#21858=CARTESIAN_POINT ( 'NONE',  ( 27.58086407627208203, -292.4444518529926427, -236.7612173134350826 ) ) ;
#21859=CARTESIAN_POINT ( 'NONE',  ( -109.8097070444448349, -289.7315620404317542, -296.3631503910306151 ) ) ;
#21861=CARTESIAN_POINT ( 'NONE',  ( -6.055683107054672831, -293.2236937891813113, -340.0733223194781658 ) ) ;
#21862=CARTESIAN_POINT ( 'NONE',  ( -96.39396084986779556, -283.5666449385989836, -226.0974656190506948 ) ) ;
#21863=CARTESIAN_POINT ( 'NONE',  ( -11.85806695174627379, -294.2477261964335753, -200.5822373150134581 ) ) ;
#21864=CARTESIAN_POINT ( 'NONE',  ( -33.45349800470193458, -284.3173967799020829, -343.7640020148577378 ) ) ;
#21865=CARTESIAN_POINT ( 'NONE',  ( -108.5756480587519519, -291.1291894498090187, -298.9713412359251379 ) ) ;
#21866=CARTESIAN_POINT ( 'NONE',  ( 33.81890197185039426, -281.8262572961833143, -253.8034263965678292 ) ) ;
#21867=CARTESIAN_POINT ( 'NONE',  ( 38.46126848937843334, -292.2037924384628127, -258.9630470732304843 ) ) ;
#21869=CARTESIAN_POINT ( 'NONE',  ( -65.37855612990146881, -290.2121659811692211, -341.9581913109369680 ) ) ;
#21870=CARTESIAN_POINT ( 'NONE',  ( 20.53075473645706595, -288.7311126993523658, -321.0791517388142893 ) ) ;
#21871=CARTESIAN_POINT ( 'NONE',  ( -19.81791149459072443, -286.4504710328173473, -199.4956338847855477 ) ) ;
#21873=DIRECTION ( 'NONE',  ( 0.000000000000000000, 0.000000000000000000, -1.000000000000000000 ) ) ;
#21874=CARTESIAN_POINT ( 'NONE',  ( 5.928315720354267349, -296.3330965711999170, -332.6183948048196157 ) ) ;
#21876=CARTESIAN_POINT ( 'NONE',  ( -97.03326717451039940, -294.5914587491922134, -318.2380484803269383 ) ) ;
#21878=CARTESIAN_POINT ( 'NONE',  ( -108.5155169900114913, -277.8378125780733967, -253.1072418331954452 ) ) ;
#21879=CARTESIAN_POINT ( 'NONE',  ( -106.7849836629186342, -272.4847827561006852, -237.2377534953233180 ) ) ;
#21880=CARTESIAN_POINT ( 'NONE',  ( -45.18357789638266553, -293.6329974703625112, -343.6869863054122902 ) ) ;
#21881=CARTESIAN_POINT ( 'NONE',  ( 34.81675088510943539, -277.0973894392573129, -253.8384461560079899 ) ) ;
#21882=CARTESIAN_POINT ( 'NONE',  ( -86.10397844571753012, -271.5075962882691556, -214.3184720172129119 ) ) ;
#21883=CARTESIAN_POINT ( 'NONE',  ( 35.10340015363704680, -294.6016065963480060, -258.4996747531023402 ) ) ;
#21884=CARTESIAN_POINT ( 'NONE',  ( -39.68520223580119932, -296.1619122369672255, -343.6452470055027106 ) ) ;
#21886=CARTESIAN_POINT ( 'NONE',  ( -92.30437754061871658, -295.2687883221487368, -219.0101579970234127 ) ) ;
#21887=CARTESIAN_POINT ( 'NONE',  ( -35.83896356287420559, -298.7219130958772553, -193.4628888928136519 ) ) ;
#21888=CARTESIAN_POINT ( 'NONE',  ( -57.42091067607932331, -275.7932986017389680, -198.0447492931461397 ) ) ;
#21889=CARTESIAN_POINT ( 'NONE',  ( -97.53549015575222825, -290.9137989181900821, -312.0978437768437743 ) ) ;
#21890=CARTESIAN_POINT ( 'NONE',  ( 10.30852592983934635, -294.7062326978360716, -325.6923337952869701 ) ) ;
#21891=CARTESIAN_POINT ( 'NONE',  ( -98.30395453017600005, -279.9312396835658774, -314.6776356712832126 ) ) ;
#21892=CARTESIAN_POINT ( 'NONE',  ( -111.2502540149691868, -277.4866846746982674, -250.5413148976952016 ) ) ;
#21893=CARTESIAN_POINT ( 'NONE',  ( -34.49106612597262966, -282.3657913624235221, -347.2063304075936117 ) ) ;
#21894=CARTESIAN_POINT ( 'NONE',  ( 34.62927384755150229, -274.5576514632986118, -243.2780662459047676 ) ) ;
#21895=CARTESIAN_POINT ( 'NONE',  ( -67.03176417578455926, -278.0692872619824811, -200.1831975705065361 ) ) ;
#21896=CARTESIAN_POINT ( 'NONE',  ( -66.62418970945078911, -277.6693198032149894, -201.1327695089344445 ) ) ;
#21897=CARTESIAN_POINT ( 'NONE',  ( -95.67031176573394191, -295.8620059351299574, -225.6302553106916662 ) ) ;
#21898=CARTESIAN_POINT ( 'NONE',  ( 35.37472182365043238, -277.3157794448280811, -251.9432563880057501 ) ) ;
#21900=CARTESIAN_POINT ( 'NONE',  ( -68.91059120213252243, -289.6592936070547921, -201.9233172620456287 ) ) ;
#21901=CARTESIAN_POINT ( 'NONE',  ( -73.17386796344683830, -289.5138142485358799, -338.5305202638644460 ) ) ;
#21902=CARTESIAN_POINT ( 'NONE',  ( 24.61856256205270910, -276.9766916708151143, -227.7830066726236851 ) ) ;
#21903=CARTESIAN_POINT ( 'NONE',  ( -93.49924585855379178, -271.2433656042375674, -220.6486375772183806 ) ) ;
#21904=CARTESIAN_POINT ( 'NONE',  ( -87.63651115912733758, -284.5681281219980292, -212.1994581078369890 ) ) ;
#21906=CARTESIAN_POINT ( 'NONE',  ( -46.98109279403942651, -283.9296925360795854, -195.9317964296643879 ) ) ;
#21908=CARTESIAN_POINT ( 'NONE',  ( -1.047045556708394054, -291.3402470497297259, -206.5513545429250826 ) ) ;
#21909=CARTESIAN_POINT ( 'NONE',  ( -97.56320844032468642, -283.2889362272579206, -226.9316606630473245 ) ) ;
#21912=CARTESIAN_POINT ( 'NONE',  ( -6.423100804331541624, -290.4580877275811304, -202.0307377113255143 ) ) ;
#21913=CARTESIAN_POINT ( 'NONE',  ( -81.17921619897602170, -282.1154690976378561, -332.8832359042157236 ) ) ;
#21914=CARTESIAN_POINT ( 'NONE',  ( -13.50796996540874062, -278.3377598353536655, -340.2603431134395464 ) ) ;
#21915=CARTESIAN_POINT ( 'NONE',  ( -70.90616520926563737, -286.8241850355483962, -201.5030363627239467 ) ) ;
#21916=CARTESIAN_POINT ( 'NONE',  ( 21.96169243167951279, -288.1472345162380861, -312.9299755066104467 ) ) ;
#21917=CARTESIAN_POINT ( 'NONE',  ( -110.7547565814043509, -279.9017681422110400, -276.1431078962623928 ) ) ;
#21918=CARTESIAN_POINT ( 'NONE',  ( -85.20317312053103365, -278.5357210789944133, -325.7624850049226666 ) ) ;
#21919=CARTESIAN_POINT ( 'NONE',  ( -111.0379955077829521, -286.7345149892592531, -256.1671586330120931 ) ) ;
#21920=ORIENTED_EDGE ( 'NONE', *, *, #58044, .T. ) ;
#21921=CARTESIAN_POINT ( 'NONE',  ( -111.6215059007110710, -296.6417751110072345, -249.8783965832315630 ) ) ;
#21922=CARTESIAN_POINT ( 'NONE',  ( 36.76002388333314030, -289.6479998257419197, -279.3489597991003848 ) ) ;
#21925=CARTESIAN_POINT ( 'NONE',  ( -2.659677404128715672, -288.9805209788416391, -198.2697987213421698 ) ) ;
#21927=CARTESIAN_POINT ( 'NONE',  ( 34.70298730845203039, -291.6340781659510526, -245.3818534925929953 ) ) ;
#21928=CARTESIAN_POINT ( 'NONE',  ( 34.66943075076979852, -288.8676928704126112, -254.7052952924910301 ) ) ;
#21930=CARTESIAN_POINT ( 'NONE',  ( -14.01040691084398127, -282.1190220573713532, -200.0671765169583125 ) ) ;
#21931=CARTESIAN_POINT ( 'NONE',  ( 35.39248464043736675, -289.2741619049751876, -293.7778781920334836 ) ) ;
#21932=CARTESIAN_POINT ( 'NONE',  ( 37.62841742264924960, -289.0593618526050363, -285.6182392299298272 ) ) ;
#21933=CARTESIAN_POINT ( 'NONE',  ( -97.51144499442702340, -285.9409997001773149, -315.1339049659738407 ) ) ;
#21934=CARTESIAN_POINT ( 'NONE',  ( -107.5752326963193468, -278.3142554721811166, -302.0542940243235535 ) ) ;
#21936=CARTESIAN_POINT ( 'NONE',  ( 3.429328500152924786, -292.5888866159577333, -334.0390385296740305 ) ) ;
#21937=CARTESIAN_POINT ( 'NONE',  ( 37.98511011499103773, -281.1850234610770940, -254.3333312591005608 ) ) ;
#21938=CARTESIAN_POINT ( 'NONE',  ( -18.98878012808116011, -276.1511814444486959, -198.3770370581977147 ) ) ;
#21940=CARTESIAN_POINT ( 'NONE',  ( -110.4683760289727132, -287.2662352645559167, -253.7030783399848985 ) ) ;
#21941=CARTESIAN_POINT ( 'NONE',  ( -69.67987507718078177, -271.8721873071249320, -201.5848681080314577 ) ) ;
#21943=CARTESIAN_POINT ( 'NONE',  ( -107.6758518614634994, -278.3215429566780017, -250.5386277043601808 ) ) ;
#21944=CARTESIAN_POINT ( 'NONE',  ( -6.719263047997801941, -277.8640867952962594, -340.5912196087805910 ) ) ;
#21945=CARTESIAN_POINT ( 'NONE',  ( -37.16628714595570671, -299.4796723730357257, -196.7689696390240215 ) ) ;
#21946=CARTESIAN_POINT ( 'NONE',  ( -111.6502332804678872, -283.3684833516811068, -289.6762363067020374 ) ) ;
#21947=CARTESIAN_POINT ( 'NONE',  ( -98.16910604117829564, -291.7325559568712379, -312.5497204895880827 ) ) ;
#21948=CARTESIAN_POINT ( 'NONE',  ( -96.81822016697913114, -298.7187174500181186, -222.5568156675638249 ) ) ;
#21949=CARTESIAN_POINT ( 'NONE',  ( -112.9998085514543362, -297.9090507434886490, -258.2837793831055819 ) ) ;
#21950=CARTESIAN_POINT ( 'NONE',  ( 32.30085678040687469, -295.9111951916754606, -297.8881008007910509 ) ) ;
#21951=CARTESIAN_POINT ( 'NONE',  ( -56.82003616209836849, -281.3037452256640449, -342.6149957259304983 ) ) ;
#21952=CARTESIAN_POINT ( 'NONE',  ( -114.3690162180213434, -290.2080735928898321, -271.2242829903925099 ) ) ;
#21953=CARTESIAN_POINT ( 'NONE',  ( -35.32108957620051370, -272.0977164895359124, -195.7308805423097056 ) ) ;
#21954=CARTESIAN_POINT ( 'NONE',  ( -64.28360000871253987, -287.3065295211272314, -199.0689474654559206 ) ) ;
#21955=CARTESIAN_POINT ( 'NONE',  ( -92.65396864172502944, -288.7887316762374326, -318.5491472107341338 ) ) ;
#21956=CARTESIAN_POINT ( 'NONE',  ( -62.24311029045266253, -183.5800764965874521, -362.2538417114638492 ) ) ;
#21957=VERTEX_POINT ( 'NONE', #28177 ) ;
#21958=CARTESIAN_POINT ( 'NONE',  ( -92.37500651719146560, -289.8588878371484157, -217.2769819469097001 ) ) ;
#21959=CARTESIAN_POINT ( 'NONE',  ( -13.28491122373756639, -288.3976034221225291, -339.3057217913893737 ) ) ;
#21961=CARTESIAN_POINT ( 'NONE',  ( -95.59082690957457373, -286.3083017322741739, -220.3962678645182223 ) ) ;
#21962=CARTESIAN_POINT ( 'NONE',  ( -3.853989628314376858, -276.9308503817231326, -335.2507221756457625 ) ) ;
#21963=CARTESIAN_POINT ( 'NONE',  ( 38.02402953234110328, -292.2942411240479714, -256.1660729583650777 ) ) ;
#21964=CARTESIAN_POINT ( 'NONE',  ( -33.05612389545042618, -283.6509437124044553, -347.1527912793576434 ) ) ;
#21966=CARTESIAN_POINT ( 'NONE',  ( -33.07795995679678214, -284.5195121670786307, -346.5615894048157202 ) ) ;
#21967=CARTESIAN_POINT ( 'NONE',  ( -101.3991883220381709, -284.3223244763121329, -313.1461265848306539 ) ) ;
#21968=CARTESIAN_POINT ( 'NONE',  ( 35.54070384599518917, -281.8261008851792440, -265.8619316496205442 ) ) ;
#21969=CARTESIAN_POINT ( 'NONE',  ( 190.0322693938271925, 271.3142028313234277, -139.6664869709919969 ) ) ;
#21970=CARTESIAN_POINT ( 'NONE',  ( -114.3576356501603613, -272.6364962766734834, -270.3621918850458883 ) ) ;
#21971=CARTESIAN_POINT ( 'NONE',  ( 4.795094255471728850, -58.70174775560354874, -351.2244798983953160 ) ) ;
#21972=CARTESIAN_POINT ( 'NONE',  ( -36.72445948530067739, -273.2572677171451687, -197.1898020014760391 ) ) ;
#21973=CARTESIAN_POINT ( 'NONE',  ( -32.02302797092954023, -294.4944296402143209, -347.1287665616297318 ) ) ;
#21974=CARTESIAN_POINT ( 'NONE',  ( -38.10613583871115395, -140.5925546180554306, -361.3186870867007201 ) ) ;
#21975=CARTESIAN_POINT ( 'NONE',  ( -41.15134768539596166, -272.6901124389207212, -193.8972504864477457 ) ) ;
#21976=CARTESIAN_POINT ( 'NONE',  ( -111.6105399639294262, -298.4337476957007311, -268.7289868583806083 ) ) ;
#21977=CARTESIAN_POINT ( 'NONE',  ( -15.69048711159072518, -290.0813920908785235, -340.6458390684238111 ) ) ;
#21979=CARTESIAN_POINT ( 'NONE',  ( -65.50597995382588579, -296.3527593804980711, -341.7867340172563786 ) ) ;
#21980=CARTESIAN_POINT ( 'NONE',  ( -17.16089001868551378, -286.8120092155866701, -200.0891174969902124 ) ) ;
#21981=CARTESIAN_POINT ( 'NONE',  ( -66.09850452020098999, -272.6048492024476104, -199.2517268216630555 ) ) ;
#21982=CARTESIAN_POINT ( 'NONE',  ( 30.76395526835187155, -294.8149432394591827, -305.9388992938806382 ) ) ;
#21983=CARTESIAN_POINT ( 'NONE',  ( 17.52206569711325201, -294.7862885207600812, -324.3766276341613093 ) ) ;
#21984=CARTESIAN_POINT ( 'NONE',  ( -109.4187653402672566, -290.5651503373185847, -282.0111010213127543 ) ) ;
#21986=CARTESIAN_POINT ( 'NONE',  ( -98.41780915115799644, -275.0749542572610835, -225.7881107299815540 ) ) ;
#21987=CARTESIAN_POINT ( 'NONE',  ( 36.90418193689895077, -274.1099094640603084, -251.5048798565963182 ) ) ;
#21990=CARTESIAN_POINT ( 'NONE',  ( -110.6099939170696729, -277.7624205208140893, -294.0121355127848801 ) ) ;
#21991=CARTESIAN_POINT ( 'NONE',  ( 29.82248366146323093, -273.5426821367229309, -239.6529016023408474 ) ) ;
#21992=CARTESIAN_POINT ( 'NONE',  ( -109.8907022209534432, -273.7747057093094440, -259.4843535055481425 ) ) ;
#21993=CARTESIAN_POINT ( 'NONE',  ( 9.626830515565528046, -275.6579096443498429, -214.1042775299272023 ) ) ;
#21994=CARTESIAN_POINT ( 'NONE',  ( -104.7209098712788062, -274.7727698912561891, -235.1187653583429267 ) ) ;
#21996=CARTESIAN_POINT ( 'NONE',  ( 34.48702409058480356, -273.8648720569635771, -293.1435932646288052 ) ) ;
#21997=CARTESIAN_POINT ( 'NONE',  ( -53.16336738562419129, -295.9116935886879673, -341.7824076697121995 ) ) ;
#21998=CARTESIAN_POINT ( 'NONE',  ( -28.10036709552414891, -294.1692172851983287, -195.7123010753824417 ) ) ;
#21999=CARTESIAN_POINT ( 'NONE',  ( 35.06618330939426187, -291.9541002186154515, -257.1580441115829672 ) ) ;
#22001=CARTESIAN_POINT ( 'NONE',  ( -107.3657186184687049, -279.4537168240839264, -238.3555003850097762 ) ) ;
#22002=CARTESIAN_POINT ( 'NONE',  ( 35.58685022111462359, -275.6631082466149110, -266.1368552448271316 ) ) ;
#22004=CARTESIAN_POINT ( 'NONE',  ( -98.93717572235878777, -283.8447771984256747, -224.8945107096624554 ) ) ;
#22005=CARTESIAN_POINT ( 'NONE',  ( -109.0714872958044452, -298.8435117787939248, -247.7191634588921545 ) ) ;
#22007=CARTESIAN_POINT ( 'NONE',  ( 7.032963811566120604, -285.8709348744963563, -212.1293195123068642 ) ) ;
#22008=CARTESIAN_POINT ( 'NONE',  ( -111.1810247554213618, -276.7168675514026859, -276.1359333804008998 ) ) ;
#22009=CARTESIAN_POINT ( 'NONE',  ( -97.37683044680099442, -276.5371545943185652, -312.9407125811584365 ) ) ;
#22010=CARTESIAN_POINT ( 'NONE',  ( -111.9026023280103743, -286.6622385385496727, -261.8000237563322798 ) ) ;
#22011=CARTESIAN_POINT ( 'NONE',  ( -13.64274970330133385, -277.9427708373137307, -339.8802981559256864 ) ) ;
#22013=CARTESIAN_POINT ( 'NONE',  ( 27.82902674743269955, -273.4300503527801425, -230.7732843994919278 ) ) ;
#22014=CARTESIAN_POINT ( 'NONE',  ( -5.270814052453546950, -275.1371349643871440, -204.6559447509872598 ) ) ;
#22015=CARTESIAN_POINT ( 'NONE',  ( -25.70513905364731500, -282.2002419138664209, -196.1006381123897881 ) ) ;
#22017=CARTESIAN_POINT ( 'NONE',  ( 7.107540306442703404, -290.3725985241591729, -331.5286751730623109 ) ) ;
#22018=CARTESIAN_POINT ( 'NONE',  ( -15.38973508845747418, -290.3360127033584490, -198.5919381762314799 ) ) ;
#22019=CARTESIAN_POINT ( 'NONE',  ( 82.17294390126060932, -297.6627425910190823, -196.0436438549623972 ) ) ;
#22020=CARTESIAN_POINT ( 'NONE',  ( -92.37641378831345662, -271.9282414246493431, -221.6535849807605416 ) ) ;
#22021=CARTESIAN_POINT ( 'NONE',  ( -109.6248522415808111, -288.9118388446353265, -253.3938847739868265 ) ) ;
#22022=CARTESIAN_POINT ( 'NONE',  ( -96.12512592106646991, -239.9971452530988358, -342.0757611934672582 ) ) ;
#22023=CARTESIAN_POINT ( 'NONE',  ( -63.76076227538455754, -295.7076995178259722, -200.1133488993579306 ) ) ;
#22024=CARTESIAN_POINT ( 'NONE',  ( -95.87181665151224763, -288.3670067755102195, -319.3398762303747276 ) ) ;
#22025=CARTESIAN_POINT ( 'NONE',  ( 14.50101288419562451, -283.9084437342924616, -322.9571185482197961 ) ) ;
#22026=CARTESIAN_POINT ( 'NONE',  ( -75.57718084624754340, -283.7896530176758461, -204.6345468768586215 ) ) ;
#22027=CARTESIAN_POINT ( 'NONE',  ( -69.24835110941772598, -284.9056381947443697, -336.6874766743412692 ) ) ;
#22028=CARTESIAN_POINT ( 'NONE',  ( -91.77836989261311373, -284.6567485394690493, -319.2599281127729682 ) ) ;
#22029=CARTESIAN_POINT ( 'NONE',  ( -87.57225847614320458, -293.3348882185210869, -214.1890803815650486 ) ) ;
#22030=CARTESIAN_POINT ( 'NONE',  ( 26.12473061240615735, -275.3100814072876688, -226.7745094584619778 ) ) ;
#22031=CARTESIAN_POINT ( 'NONE',  ( -96.32387468291227606, -289.2767128729589672, -223.1338240985211598 ) ) ;
#22032=CARTESIAN_POINT ( 'NONE',  ( -42.80616938195925059, -277.1193197404836042, -347.1669743723785473 ) ) ;
#22033=CARTESIAN_POINT ( 'NONE',  ( -3.570450188973522287, -296.5841228840620261, -336.9438156009522913 ) ) ;
#22035=CARTESIAN_POINT ( 'NONE',  ( -110.4542110544635705, -292.8376638359844719, -287.0812184334320705 ) ) ;
#22036=CARTESIAN_POINT ( 'NONE',  ( -3.408475872029683273, -281.2791896537789285, -335.5655513260788894 ) ) ;
#22037=CARTESIAN_POINT ( 'NONE',  ( -110.6088843885063966, -276.7671167839473583, -253.5698064723128198 ) ) ;
#22038=CARTESIAN_POINT ( 'NONE',  ( -107.4329089919810087, -271.4213121827540931, -240.0625193506001267 ) ) ;
#22039=CARTESIAN_POINT ( 'NONE',  ( 19.25525026875159185, -275.5551475449715895, -316.6483004899915272 ) ) ;
#22040=CARTESIAN_POINT ( 'NONE',  ( -47.10530543855251295, -293.4460041974173237, -197.3174340477686428 ) ) ;
#22041=CARTESIAN_POINT ( 'NONE',  ( 35.13889872392667968, -294.3555155387959417, -259.8744007521112280 ) ) ;
#22042=CARTESIAN_POINT ( 'NONE',  ( 38.65307184076674218, -295.0839210904373431, -278.8115329236394473 ) ) ;
#22043=CARTESIAN_POINT ( 'NONE',  ( 33.99688223763389061, -294.5132154905840025, -242.5723492517441002 ) ) ;
#22044=CARTESIAN_POINT ( 'NONE',  ( -70.93268884922579787, -295.3415863591967536, -335.1874892885591066 ) ) ;
#22045=CARTESIAN_POINT ( 'NONE',  ( -45.55689817865564351, -291.1564417862485925, -344.9098347303642527 ) ) ;
#22046=CARTESIAN_POINT ( 'NONE',  ( -21.72391478033941681, -283.0239529526014053, -345.7606192097987901 ) ) ;
#22047=CARTESIAN_POINT ( 'NONE',  ( -29.93567114496962134, -272.2845364145052258, -194.9591537205789109 ) ) ;
#22048=CARTESIAN_POINT ( 'NONE',  ( 30.13258433355151666, -286.9037822666161901, -233.1530278623632739 ) ) ;
#22049=CARTESIAN_POINT ( 'NONE',  ( -69.94762602334739654, -279.4635573971074223, -337.5221219412450182 ) ) ;
#22051=CARTESIAN_POINT ( 'NONE',  ( -74.91024307277865546, -284.3346417672588586, -207.3076875773342351 ) ) ;
#22052=CARTESIAN_POINT ( 'NONE',  ( -37.52300738869169550, -287.0542291604591014, -345.3736350570965215 ) ) ;
#22053=CARTESIAN_POINT ( 'NONE',  ( -74.38302801447568413, -277.7045581109323962, -204.2684140755524425 ) ) ;
#22054=CARTESIAN_POINT ( 'NONE',  ( 24.80950920047307307, -22.49099280560490399, -345.4124233396505019 ) ) ;
#22055=CARTESIAN_POINT ( 'NONE',  ( -99.65853333932143698, -284.5860523897389953, -232.1255109798987348 ) ) ;
#22056=CARTESIAN_POINT ( 'NONE',  ( 22.55518240935465712, -282.1143248949463782, -222.5870271099866500 ) ) ;
#22057=CARTESIAN_POINT ( 'NONE',  ( 7.786474974902612978, -287.5116530156381032, -332.5255180798272931 ) ) ;
#22058=CARTESIAN_POINT ( 'NONE',  ( -112.2139773211968929, -280.3321424147909511, -256.1285220388277253 ) ) ;
#22059=CARTESIAN_POINT ( 'NONE',  ( -95.76171409509073840, -279.1972377115771451, -319.7817401263760075 ) ) ;
#22060=CARTESIAN_POINT ( 'NONE',  ( -27.55627358187902942, -280.0131043519170930, -197.9687530606426833 ) ) ;
#22061=CARTESIAN_POINT ( 'NONE',  ( -90.42928514432774989, -275.2758126436453949, -217.8867897925246098 ) ) ;
#22062=CARTESIAN_POINT ( 'NONE',  ( 28.05235832175989330, -293.0192288351423713, -229.6079759649919367 ) ) ;
#22063=CARTESIAN_POINT ( 'NONE',  ( 29.69408463706439250, -286.0072294040658107, -303.1947952131019406 ) ) ;
#22065=CARTESIAN_POINT ( 'NONE',  ( -44.83882950444907323, -293.5590148283880580, -194.4784513648361894 ) ) ;
#22066=CARTESIAN_POINT ( 'NONE',  ( -82.56124162891731544, -294.6066306310773371, -328.1269677451817302 ) ) ;
#22067=CARTESIAN_POINT ( 'NONE',  ( 35.72912095381111186, -293.2241855123219807, -270.7642741458744808 ) ) ;
#22068=CARTESIAN_POINT ( 'NONE',  ( -99.78737868035983638, -292.2238421941131605, -225.8411253914347583 ) ) ;
#22069=CARTESIAN_POINT ( 'NONE',  ( 33.42427542132536900, -282.4458356901552634, -288.7431960585911952 ) ) ;
#22070=CARTESIAN_POINT ( 'NONE',  ( -35.82189367916155476, -296.9910956121629511, -193.6704985816411408 ) ) ;
#22071=CARTESIAN_POINT ( 'NONE',  ( -5.660901615161487044, -289.2977413021542930, -340.4299398119526359 ) ) ;
#22072=CARTESIAN_POINT ( 'NONE',  ( -49.91227963785794230, -281.3503251986054465, -345.1288282643165530 ) ) ;
#22073=CARTESIAN_POINT ( 'NONE',  ( 5.549062532552957450, -288.8216608659247981, -334.2839368334825281 ) ) ;
#22074=CARTESIAN_POINT ( 'NONE',  ( -38.62953629823759627, -286.3688797193307209, -197.3388459742041050 ) ) ;
#22076=CARTESIAN_POINT ( 'NONE',  ( -108.0872568736431276, -260.2256227728311160, -316.3845286481523544 ) ) ;
#22077=CARTESIAN_POINT ( 'NONE',  ( -105.4589550887750988, -260.1083542854994448, -315.4719013409242052 ) ) ;
#22078=CARTESIAN_POINT ( 'NONE',  ( -57.14712512772582897, -278.9871598176096086, -199.9313879881560183 ) ) ;
#22079=CARTESIAN_POINT ( 'NONE',  ( -79.22023687147216719, -278.3923204521280468, -210.1912398614051085 ) ) ;
#22080=CARTESIAN_POINT ( 'NONE',  ( 7.226205466581010484, -274.3075671297090139, -207.5306920235136658 ) ) ;
#22081=CARTESIAN_POINT ( 'NONE',  ( -104.6257879195275109, -262.2290025098591855, -316.4541994228543444 ) ) ;
#22082=CARTESIAN_POINT ( 'NONE',  ( -110.7659831213586301, -277.3941555624001012, -249.2073722050611195 ) ) ;
#22083=CARTESIAN_POINT ( 'NONE',  ( -38.94513464922362544, -281.0924407706675083, -345.0014707077602907 ) ) ;
#22084=CARTESIAN_POINT ( 'NONE',  ( -41.86256625807790499, -296.8683808095737504, -346.2648876686359358 ) ) ;
#22085=CARTESIAN_POINT ( 'NONE',  ( -95.16693801237609307, -291.6726911288322412, -225.7043121688516010 ) ) ;
#22086=CARTESIAN_POINT ( 'NONE',  ( -96.17309108007361829, -288.6226318876221626, -314.4288160037789339 ) ) ;
#22087=CARTESIAN_POINT ( 'NONE',  ( 11.71427823649671573, -275.3638067033971311, -211.0734894895038565 ) ) ;
#22088=CARTESIAN_POINT ( 'NONE',  ( -98.73215289570036646, -296.1710757018130380, -309.9532392955114233 ) ) ;
#22092=CARTESIAN_POINT ( 'NONE',  ( -108.2632307133195297, -280.8097462131869406, -244.1436519893845229 ) ) ;
#22093=CARTESIAN_POINT ( 'NONE',  ( -43.79193168206481346, -281.0485387096636600, -197.2858770015112668 ) ) ;
#22094=CARTESIAN_POINT ( 'NONE',  ( -88.26912268362117686, -281.1104411273269648, -213.9663341499709190 ) ) ;
#22095=CARTESIAN_POINT ( 'NONE',  ( 17.77405764104748798, -281.2967919033375779, -318.5862327476772862 ) ) ;
#22096=CARTESIAN_POINT ( 'NONE',  ( -35.35239066189981827, -272.5574123695898834, -196.6820132493316464 ) ) ;
#22099=CARTESIAN_POINT ( 'NONE',  ( 38.05831960672234970, -276.1695162504791483, -255.5626097816515596 ) ) ;
#22102=CARTESIAN_POINT ( 'NONE',  ( 22.85890001193301657, -276.9416516776275898, -225.6298269853682825 ) ) ;
#22103=CARTESIAN_POINT ( 'NONE',  ( -75.06125039791029963, -276.1192420736601889, -336.8129187151195083 ) ) ;
#22105=CARTESIAN_POINT ( 'NONE',  ( -87.21367931486913960, -285.7225291876022766, -326.9214104897814650 ) ) ;
#22106=CARTESIAN_POINT ( 'NONE',  ( 16.86468766532961183, -292.0461569398232768, -221.1515885977380549 ) ) ;
#22108=CARTESIAN_POINT ( 'NONE',  ( 2.695029425714173144, -285.9229736202519234, -204.7076864414023873 ) ) ;
#22109=CARTESIAN_POINT ( 'NONE',  ( -89.62578124426643456, -282.0411623410666948, -322.8196108243830622 ) ) ;
#22110=CARTESIAN_POINT ( 'NONE',  ( -26.67516214311025280, -281.4886774185390550, -343.2249162273571415 ) ) ;
#22111=CARTESIAN_POINT ( 'NONE',  ( -23.97822540288576576, -284.0827161764458424, -342.5313891958876980 ) ) ;
#22112=CARTESIAN_POINT ( 'NONE',  ( -32.77816706851746176, -272.1094782177806337, -195.4872723704287978 ) ) ;
#22113=CARTESIAN_POINT ( 'NONE',  ( -110.9431073469294802, -283.2039273498729699, -250.4329958359720649 ) ) ;
#22114=CARTESIAN_POINT ( 'NONE',  ( -30.74092480879376765, -296.9688542094201580, -345.0700894240405319 ) ) ;
#22115=CARTESIAN_POINT ( 'NONE',  ( -89.65000708968557319, -280.2336095024909355, -219.0325341674079596 ) ) ;
#22116=CARTESIAN_POINT ( 'NONE',  ( -13.31443234037744183, -288.3636626828387648, -199.1380962288147884 ) ) ;
#22119=CARTESIAN_POINT ( 'NONE',  ( 21.18703404804402979, -296.1261458901512924, -318.1695276976710147 ) ) ;
#22121=CARTESIAN_POINT ( 'NONE',  ( -109.7578302270225663, -276.3010762859791498, -289.8778992926926890 ) ) ;
#22122=CARTESIAN_POINT ( 'NONE',  ( 20.44469823219483118, -287.4361421746965561, -321.0256893788560433 ) ) ;
#22123=CARTESIAN_POINT ( 'NONE',  ( 32.28813893876350960, -292.2756925488212119, -294.9706231266723080 ) ) ;
#22124=CARTESIAN_POINT ( 'NONE',  ( -41.90381846841076197, -275.7956293297857542, -343.7252176699694246 ) ) ;
#22125=CARTESIAN_POINT ( 'NONE',  ( -94.04089835848893131, -294.0219229490073189, -318.2981056590870708 ) ) ;
#22126=CARTESIAN_POINT ( 'NONE',  ( -100.1416392193741558, -292.3895593927554160, -232.1850636094812046 ) ) ;
#22127=CARTESIAN_POINT ( 'NONE',  ( -37.30987171927208124, -285.5519495502701943, -345.3611179825600175 ) ) ;
#22128=CARTESIAN_POINT ( 'NONE',  ( -2.303234979380001768, -293.0768387492785223, -338.1476484627474406 ) ) ;
#22129=CARTESIAN_POINT ( 'NONE',  ( -99.50476808335670853, -291.6080240857183981, -310.1379126885870505 ) ) ;
#22130=CARTESIAN_POINT ( 'NONE',  ( -111.3254551891057247, -289.0116684509216611, -253.0297012861432790 ) ) ;
#22131=CARTESIAN_POINT ( 'NONE',  ( -26.36925067790773625, -290.3352001329694190, -343.1791956797229091 ) ) ;
#22133=CARTESIAN_POINT ( 'NONE',  ( -95.07168560295637860, -290.7229380147977054, -315.3241013266531922 ) ) ;
#22135=CARTESIAN_POINT ( 'NONE',  ( -51.59629486533960119, -290.4356736415537625, -345.6260849087109364 ) ) ;
#22136=CARTESIAN_POINT ( 'NONE',  ( -110.1354556039400592, -276.8220739507396502, -250.8312221900138468 ) ) ;
#22137=CARTESIAN_POINT ( 'NONE',  ( -103.3956343133897917, -279.4021852757245483, -230.7274491460136687 ) ) ;
#22138=CARTESIAN_POINT ( 'NONE',  ( 35.30914228429821122, -280.8960175089619611, -244.7539119773361165 ) ) ;
#22139=CARTESIAN_POINT ( 'NONE',  ( 30.63307416003257089, -285.1354721084101698, -238.6683631933582035 ) ) ;
#22141=CARTESIAN_POINT ( 'NONE',  ( -3.071879666528419595, -280.7340358851059250, -336.2270467589209488 ) ) ;
#22142=CARTESIAN_POINT ( 'NONE',  ( -106.0825702173391818, -282.9460941949111543, -240.2364737273184119 ) ) ;
#22144=CARTESIAN_POINT ( 'NONE',  ( -104.3758221352403126, -276.5559851423716964, -306.8184113241194382 ) ) ;
#22145=CARTESIAN_POINT ( 'NONE',  ( -111.9217889233537875, -283.2474106860418601, -288.2857971699683048 ) ) ;
#22146=CARTESIAN_POINT ( 'NONE',  ( -103.3551642575919516, -273.7806015108240558, -238.8202828630230101 ) ) ;
#22147=CARTESIAN_POINT ( 'NONE',  ( -106.4670620156734060, -292.4950863085143737, -244.3678915975998507 ) ) ;
#22148=CARTESIAN_POINT ( 'NONE',  ( -93.72285049825497083, -274.6844223999264614, -218.7688147723552277 ) ) ;
#22149=CARTESIAN_POINT ( 'NONE',  ( 34.14291645092834671, -275.0215539068581734, -255.3991503462194146 ) ) ;
#22150=CARTESIAN_POINT ( 'NONE',  ( -96.33113357565775914, -297.9165606087130413, -316.6779334472983578 ) ) ;
#22151=CARTESIAN_POINT ( 'NONE',  ( -9.561351126600849071, -288.8656785706443202, -342.1751292468177326 ) ) ;
#22152=CARTESIAN_POINT ( 'NONE',  ( 36.58107147869814213, -279.4318331750414472, -254.6550208814402652 ) ) ;
#22153=CARTESIAN_POINT ( 'NONE',  ( 30.89990797362019848, -292.9240255349965310, -234.5800561597016838 ) ) ;
#22154=CARTESIAN_POINT ( 'NONE',  ( -38.89057644368904221, -291.0909937490118295, -197.1422035480904640 ) ) ;
#22155=CARTESIAN_POINT ( 'NONE',  ( 9.917788682466211370, -292.4014632694477882, -328.6649678520193447 ) ) ;
#22158=CARTESIAN_POINT ( 'NONE',  ( -107.8095829145748326, -290.3145046411170256, -251.0669235867877944 ) ) ;
#22160=CARTESIAN_POINT ( 'NONE',  ( -35.16695040813171147, -287.0200468475034654, -193.6141193639876974 ) ) ;
#22161=CARTESIAN_POINT ( 'NONE',  ( -82.08285599513421005, -276.9094976428775681, -214.2051214447836571 ) ) ;
#22162=CARTESIAN_POINT ( 'NONE',  ( 19.34779862607356193, -293.3174921773381811, -322.1987546065767560 ) ) ;
#22163=CARTESIAN_POINT ( 'NONE',  ( -90.08595395822472085, -285.0937366283082497, -325.8534319123103842 ) ) ;
#22164=CARTESIAN_POINT ( 'NONE',  ( -46.72276634727607103, -285.7631942962228777, -197.9156218335947415 ) ) ;
#22165=CARTESIAN_POINT ( 'NONE',  ( 18.84951794254120117, -277.7437967066101692, -318.0397795173426516 ) ) ;
#22166=CARTESIAN_POINT ( 'NONE',  ( 35.37206869002721987, -291.7905415748623454, -287.2860912335888202 ) ) ;
#22167=CARTESIAN_POINT ( 'NONE',  ( -36.96823175198149869, -296.8075223592193197, -344.3861095276251945 ) ) ;
#22168=CARTESIAN_POINT ( 'NONE',  ( 24.30962165790098695, -274.8965906410148818, -310.2824929164183914 ) ) ;
#22171=CARTESIAN_POINT ( 'NONE',  ( -37.69314251029897633, -294.7231250274949161, -347.3522466207692219 ) ) ;
#22172=CARTESIAN_POINT ( 'NONE',  ( 35.98156636610907810, -289.3023750589509291, -257.2251602155025125 ) ) ;
#22173=CARTESIAN_POINT ( 'NONE',  ( -83.98625600570882455, -296.7554854291993820, -331.3031652977419981 ) ) ;
#22174=CARTESIAN_POINT ( 'NONE',  ( -17.15167285799614660, -286.9710496297568625, -200.0497078762374201 ) ) ;
#22175=CARTESIAN_POINT ( 'NONE',  ( -89.06245291972591360, -276.8173499521330427, -327.0866320221732622 ) ) ;
#22176=CARTESIAN_POINT ( 'NONE',  ( -69.47775345365398891, -296.1154793590793588, -340.2367282493395919 ) ) ;
#22177=CARTESIAN_POINT ( 'NONE',  ( -37.52280776917235983, -287.1939510637074022, -346.1385669946510006 ) ) ;
#22178=CARTESIAN_POINT ( 'NONE',  ( -112.5835933026689304, -296.6820164107526807, -286.6215547280542637 ) ) ;
#22179=CARTESIAN_POINT ( 'NONE',  ( -49.69647704797255017, -292.2236489684635785, -198.3414022905857905 ) ) ;
#22182=CARTESIAN_POINT ( 'NONE',  ( -88.01845085740878005, -229.9137135291813365, -344.5856900491873489 ) ) ;
#22183=CARTESIAN_POINT ( 'NONE',  ( -33.77923857464701740, -287.6163341169957448, -194.1376529509589659 ) ) ;
#22184=CARTESIAN_POINT ( 'NONE',  ( 40.65961533371913106, -284.8380690714489560, -252.5904736702033802 ) ) ;
#22186=CARTESIAN_POINT ( 'NONE',  ( -113.1346158339228651, -278.0634180704651612, -257.3708633454112373 ) ) ;
#22187=CARTESIAN_POINT ( 'NONE',  ( -93.92916999590963201, -285.8714485896629185, -319.3488311274430203 ) ) ;
#22188=CARTESIAN_POINT ( 'NONE',  ( -110.1298315720598566, -282.8318573188327036, -293.6528307703787277 ) ) ;
#22189=CARTESIAN_POINT ( 'NONE',  ( -45.54495075267553261, -287.2367591935550877, -344.3477443156335767 ) ) ;
#22190=CARTESIAN_POINT ( 'NONE',  ( 37.27147938519131998, -277.2443599666023601, -257.1273687462525572 ) ) ;
#22191=CARTESIAN_POINT ( 'NONE',  ( -109.8647781493528583, -296.9224666840913187, -279.6198576391023494 ) ) ;
#22192=CARTESIAN_POINT ( 'NONE',  ( -26.14871156161469301, -293.5914854915856154, -342.9969251574776763 ) ) ;
#22193=CARTESIAN_POINT ( 'NONE',  ( -93.00570585509343857, -279.9305526717643602, -217.2300448862810640 ) ) ;
#22194=CARTESIAN_POINT ( 'NONE',  ( 15.59787931475365674, -276.2767034632022387, -320.6244339139205408 ) ) ;
#22195=CARTESIAN_POINT ( 'NONE',  ( -108.0690998730582919, -278.1449764571256651, -251.8315056525128739 ) ) ;
#22196=CARTESIAN_POINT ( 'NONE',  ( -44.02956050058333659, -275.0492799886968101, -193.9092992939274041 ) ) ;
#22197=CARTESIAN_POINT ( 'NONE',  ( -20.20859208524191075, -275.7574756614356488, -345.1682007661023022 ) ) ;
#22198=CARTESIAN_POINT ( 'NONE',  ( 84.21812867662228541, 83.45443861164879706, -302.1763853416691745 ) ) ;
#22199=CARTESIAN_POINT ( 'NONE',  ( 30.74250727900928126, -273.9665778163246159, -301.9402080428728254 ) ) ;
#22200=CARTESIAN_POINT ( 'NONE',  ( -103.3500167102587710, -298.4832830842162252, -231.7664360560755199 ) ) ;
#22203=CARTESIAN_POINT ( 'NONE',  ( -14.48261541762676430, -287.4351067973700538, -200.6538171777995387 ) ) ;
#22204=CARTESIAN_POINT ( 'NONE',  ( -60.22637820178681523, -287.5197486980457597, -197.8475513429349917 ) ) ;
#22205=CARTESIAN_POINT ( 'NONE',  ( 17.85860097880830466, -286.2184885290956231, -222.4359739960347042 ) ) ;
#22206=CARTESIAN_POINT ( 'NONE',  ( -96.23801573427232370, -277.5702114631654354, -225.8692096821175426 ) ) ;
#22207=CARTESIAN_POINT ( 'NONE',  ( -96.76874868663158225, -287.0266296698727047, -225.8718902713021350 ) ) ;
#22208=CARTESIAN_POINT ( 'NONE',  ( -108.6384978430881461, -277.2764081619799299, -251.6709374264213182 ) ) ;
#22209=CARTESIAN_POINT ( 'NONE',  ( 3.421456510655424221, -277.8064741970088107, -331.5134567606641554 ) ) ;
#22210=CARTESIAN_POINT ( 'NONE',  ( -2.890174278974634969, -275.0129076687061342, -205.9322361944807085 ) ) ;
#22211=CARTESIAN_POINT ( 'NONE',  ( 37.11482357245765940, -286.5741085521617038, -288.4230053044920510 ) ) ;
#22212=CARTESIAN_POINT ( 'NONE',  ( 36.82645904412814275, -282.1024078412224299, -250.2303356975590987 ) ) ;
#22213=CARTESIAN_POINT ( 'NONE',  ( -8.056497279534728051, -283.1711699926710253, -341.5646719540514482 ) ) ;
#22217=CARTESIAN_POINT ( 'NONE',  ( 17.76297131009744490, -290.1341867999327064, -322.3590089598238819 ) ) ;
#22218=CARTESIAN_POINT ( 'NONE',  ( -77.88933870526683734, -288.2692228764158813, -335.3011739738267352 ) ) ;
#22219=CARTESIAN_POINT ( 'NONE',  ( -4.825223653120814582, -296.2311946048604909, -339.2892929830470052 ) ) ;
#22220=CARTESIAN_POINT ( 'NONE',  ( -102.2333929932004537, -272.0727295929950742, -236.3031684576393729 ) ) ;
#22222=CARTESIAN_POINT ( 'NONE',  ( 8.796404474466545054, -292.0144727706777417, -208.7756489966121478 ) ) ;
#22223=CARTESIAN_POINT ( 'NONE',  ( 29.44641053649024443, -285.6154333585424752, -239.2153955738508841 ) ) ;
#22224=CARTESIAN_POINT ( 'NONE',  ( -44.37448219349185052, -290.2019754038470865, -196.6311454344262870 ) ) ;
#22225=CARTESIAN_POINT ( 'NONE',  ( 35.66780817446930740, -288.6584019714782698, -262.8283759998219580 ) ) ;
#22226=CARTESIAN_POINT ( 'NONE',  ( 35.77081079830085031, -289.8376638359844719, -253.6410175316879361 ) ) ;
#22227=CARTESIAN_POINT ( 'NONE',  ( 37.70171403041528890, -289.5668755362885918, -271.4949553583992383 ) ) ;
#22228=CARTESIAN_POINT ( 'NONE',  ( -108.6826151180768392, -288.8591520862484572, -246.5234751746968129 ) ) ;
#22229=CARTESIAN_POINT ( 'NONE',  ( -109.9721806977819227, -292.3114130144335263, -289.1150650117858731 ) ) ;
#22230=CARTESIAN_POINT ( 'NONE',  ( -110.5534734773341938, -285.4500233752038412, -273.6606515812145517 ) ) ;
#22231=CARTESIAN_POINT ( 'NONE',  ( -30.88085797615934780, -294.1336568521236927, -195.4211257457027102 ) ) ;
#22234=CARTESIAN_POINT ( 'NONE',  ( -64.33495462278260391, -275.6815556624387682, -199.9926242070763180 ) ) ;
#22235=CARTESIAN_POINT ( 'NONE',  ( 33.47724435056878178, -280.9918250630988723, -288.7761442953181472 ) ) ;
#22236=CARTESIAN_POINT ( 'NONE',  ( -108.9015518976414398, -282.2623234398820387, -292.8152548785163276 ) ) ;
#22237=CARTESIAN_POINT ( 'NONE',  ( -112.4494906573325608, -295.5460865157887724, -286.5777336305656036 ) ) ;
#22238=CARTESIAN_POINT ( 'NONE',  ( -13.72111821650113228, -272.6028334364460193, -200.2181060536160544 ) ) ;
#22239=CARTESIAN_POINT ( 'NONE',  ( -59.64936969553718171, -275.4231879672407786, -341.3800033185805773 ) ) ;
#22240=CARTESIAN_POINT ( 'NONE',  ( -109.0695403192397777, -297.6575303897711819, -286.3723771831532758 ) ) ;
#22242=CARTESIAN_POINT ( 'NONE',  ( -52.41151477871648723, -272.4376632742024071, -195.3971037112025897 ) ) ;
#22243=CARTESIAN_POINT ( 'NONE',  ( -111.6053022474380185, -294.9966496422327964, -254.2103682178892825 ) ) ;
#22244=CARTESIAN_POINT ( 'NONE',  ( 14.74607274401700963, -295.7263747231954767, -322.4158481592006069 ) ) ;
#22245=CARTESIAN_POINT ( 'NONE',  ( 151.9709352735115147, -299.5541904835127980, -195.3611179825600175 ) ) ;
#22246=CARTESIAN_POINT ( 'NONE',  ( -53.17438228851172255, -296.0630885945287787, -341.8409971645655219 ) ) ;
#22248=CARTESIAN_POINT ( 'NONE',  ( -110.9245596023432938, -282.3646367271575173, -286.6082592393852337 ) ) ;
#22249=CARTESIAN_POINT ( 'NONE',  ( -110.2416699368873196, -296.5017565662486163, -274.1813799991211908 ) ) ;
#22250=CARTESIAN_POINT ( 'NONE',  ( -107.0056437063501278, -284.1319971480290860, -303.1625655896975218 ) ) ;
#22251=CARTESIAN_POINT ( 'NONE',  ( -31.71858921361257799, -284.9018791663603452, -345.7246177489112142 ) ) ;
#22252=CARTESIAN_POINT ( 'NONE',  ( 26.34225995688074562, -286.6482913586738164, -227.0929448413731109 ) ) ;
#22253=CARTESIAN_POINT ( 'NONE',  ( 32.54952155606841302, -291.2035751591625399, -243.6170428255205422 ) ) ;
#22254=CARTESIAN_POINT ( 'NONE',  ( -50.90107174682299984, -279.0802838820051193, -194.7284381322464810 ) ) ;
#22255=CARTESIAN_POINT ( 'NONE',  ( -37.37352853689063181, -274.5523547857346784, -345.3611179825600175 ) ) ;
#22257=CARTESIAN_POINT ( 'NONE',  ( 30.84842715446182027, -286.7100404913146008, -297.6502300408513975 ) ) ;
#22258=CARTESIAN_POINT ( 'NONE',  ( -112.5674954545477533, -289.2843161470996165, -285.3465955838249215 ) ) ;
#22259=DIRECTION ( 'NONE',  ( 0.000000000000000000, 0.000000000000000000, 1.000000000000000000 ) ) ;
#22261=CARTESIAN_POINT ( 'NONE',  ( -109.9951378517421148, -280.2793432260988311, -246.5269591809231997 ) ) ;
#22262=CARTESIAN_POINT ( 'NONE',  ( -100.1642185272913821, -295.1319036797182207, -228.7234769323524688 ) ) ;
#22263=CARTESIAN_POINT ( 'NONE',  ( 21.34849923393327131, -280.6096557665269984, -226.8941514325418609 ) ) ;
#22264=CARTESIAN_POINT ( 'NONE',  ( -50.46543365354227717, -295.3818323735723652, -346.2884284626431963 ) ) ;
#22265=CARTESIAN_POINT ( 'NONE',  ( -112.0836304866057134, -280.4648215115045673, -277.1753842732701969 ) ) ;
#22266=CARTESIAN_POINT ( 'NONE',  ( -108.5305625601052952, -295.3841446237775017, -287.6057295929663269 ) ) ;
#22269=CARTESIAN_POINT ( 'NONE',  ( 17.04110970482810217, -284.2525407641870174, -321.5665002404175539 ) ) ;
#22271=CARTESIAN_POINT ( 'NONE',  ( -54.42813229853333468, -295.3380690714489560, -195.3538533559490702 ) ) ;
#22272=CARTESIAN_POINT ( 'NONE',  ( -32.68215819214907469, -273.3066127776787084, -193.6508797292545694 ) ) ;
#22275=CARTESIAN_POINT ( 'NONE',  ( -109.4194431664759435, -290.2318440797944845, -282.0069061936464436 ) ) ;
#22276=CARTESIAN_POINT ( 'NONE',  ( 13.80248491921587117, -282.3048035628567050, -217.2336380784568348 ) ) ;
#22277=CARTESIAN_POINT ( 'NONE',  ( -13.82964972427402195, -275.9625615892384758, -200.4066763793818495 ) ) ;
#22278=CARTESIAN_POINT ( 'NONE',  ( -0.7416024824666248572, -284.1745283448616419, -337.2105748063932538 ) ) ;
#22279=CARTESIAN_POINT ( 'NONE',  ( 28.14255930824677066, -279.8980774887751295, -237.0980804190692766 ) ) ;
#22280=CARTESIAN_POINT ( 'NONE',  ( -111.0028955777129482, -280.3702994175069989, -284.5366186649951601 ) ) ;
#22281=CARTESIAN_POINT ( 'NONE',  ( -111.8188285338560348, -272.9658686250723463, -250.6081887865874194 ) ) ;
#22282=CARTESIAN_POINT ( 'NONE',  ( -10.34562563149279768, -274.2280746691117770, -198.1918986989856251 ) ) ;
#22283=CARTESIAN_POINT ( 'NONE',  ( 11.24962205036979235, -296.2928501598140656, -326.7543587482267071 ) ) ;
#22286=CARTESIAN_POINT ( 'NONE',  ( -3.797320701080445726, -292.7540198581447726, -338.3098666641859040 ) ) ;
#22287=CARTESIAN_POINT ( 'NONE',  ( -89.28151697533074582, -272.8039718208664794, -218.9778145903534323 ) ) ;
#22288=CARTESIAN_POINT ( 'NONE',  ( -81.54464272965081761, -292.9826929803199960, -208.1613783008386633 ) ) ;
#22289=CARTESIAN_POINT ( 'NONE',  ( -54.42813229853333468, -285.7662352645560873, -345.3683826091709648 ) ) ;
#22290=CARTESIAN_POINT ( 'NONE',  ( -56.10645004155875881, -293.0208695947184765, -196.0373928719101855 ) ) ;
#22291=CARTESIAN_POINT ( 'NONE',  ( 25.79854838069763190, -290.0940410220385388, -310.5274900358434707 ) ) ;
#22292=CARTESIAN_POINT ( 'NONE',  ( -32.32241159011101672, -274.9886833397418400, -345.0771585028429058 ) ) ;
#22293=CARTESIAN_POINT ( 'NONE',  ( -90.08927113953996013, -279.7244101909936376, -322.9605495156383768 ) ) ;
#22294=CARTESIAN_POINT ( 'NONE',  ( 34.50014185757092378, -291.8851133859548668, -289.9047516695094941 ) ) ;
#22295=CARTESIAN_POINT ( 'NONE',  ( 37.45234936239019419, -283.5672578894449316, -282.5317990292687682 ) ) ;
#22296=EDGE_LOOP ( 'NONE', ( #19386, #22406, #65534, #57974 ) ) ;
#22297=CARTESIAN_POINT ( 'NONE',  ( -37.54484287652233121, -282.7215177141004574, -343.3944125572135704 ) ) ;
#22298=CARTESIAN_POINT ( 'NONE',  ( -88.73452847818180089, -280.4300808660009920, -213.4377510479040723 ) ) ;
#22299=CARTESIAN_POINT ( 'NONE',  ( -30.26692014408772025, -281.7594550964741416, -346.6366462109099871 ) ) ;
#22300=CARTESIAN_POINT ( 'NONE',  ( -5.371805337394278013, -277.5829339913037188, -340.1518483192255644 ) ) ;
#22302=CARTESIAN_POINT ( 'NONE',  ( 22.98194438822590868, -277.7021111441856647, -317.1130944794555830 ) ) ;
#22303=CARTESIAN_POINT ( 'NONE',  ( -92.05005921254146983, -292.4090924074130839, -314.0302885647153062 ) ) ;
#22305=CARTESIAN_POINT ( 'NONE',  ( -36.47938060747782174, -300.0631032878335418, -195.3608152725264517 ) ) ;
#22306=CARTESIAN_POINT ( 'NONE',  ( -48.88656166690392268, -275.2198881082672983, -344.1602806372961254 ) ) ;
#22307=CARTESIAN_POINT ( 'NONE',  ( -103.7356006400929829, -292.7977659446831353, -233.4040620059906530 ) ) ;
#22308=CARTESIAN_POINT ( 'NONE',  ( 32.84572263011548188, -293.1712189689705497, -290.8418044885499967 ) ) ;
#22309=CARTESIAN_POINT ( 'NONE',  ( 38.91511078874229668, -286.9319030931991392, -260.1422290020757373 ) ) ;
#22311=CARTESIAN_POINT ( 'NONE',  ( -39.11251653925135230, -293.6487009939369273, -346.7513693497926965 ) ) ;
#22312=CARTESIAN_POINT ( 'NONE',  ( -95.76208709428401278, -282.3238120102021185, -315.4760857406908485 ) ) ;
#22313=CARTESIAN_POINT ( 'NONE',  ( -48.21895197020887025, -291.0523013719660526, -343.8469917341868154 ) ) ;
#22314=CARTESIAN_POINT ( 'NONE',  ( -67.81691342459275518, -284.1245942245611786, -203.2644032435040060 ) ) ;
#22315=CARTESIAN_POINT ( 'NONE',  ( 5.895644465780362609, -283.7670468648700535, -329.7898611057781864 ) ) ;
#22316=CARTESIAN_POINT ( 'NONE',  ( -34.66299147064142971, -289.9605083478569441, -347.0790737262552170 ) ) ;
#22317=CARTESIAN_POINT ( 'NONE',  ( 29.02595968325211118, -281.6312435963162670, -239.6895749831276135 ) ) ;
#22318=CARTESIAN_POINT ( 'NONE',  ( 13.12265352643423810, -293.1604944259094623, -328.0626570769148884 ) ) ;
#22319=CARTESIAN_POINT ( 'NONE',  ( -3.123438277038188549, -289.4145448140963595, -339.1744766487718152 ) ) ;
#22320=CARTESIAN_POINT ( 'NONE',  ( 39.51579178095167322, -287.9876071046599009, -265.8157772788455873 ) ) ;
#22321=CARTESIAN_POINT ( 'NONE',  ( -68.77685911055181123, -285.7937025303721725, -204.4623467902760865 ) ) ;
#22324=CARTESIAN_POINT ( 'NONE',  ( 23.05883952269570614, -296.0318247268497203, -316.1003822238880616 ) ) ;
#22325=CARTESIAN_POINT ( 'NONE',  ( -44.76455706899341891, -293.8289323358789602, -346.5600922345200274 ) ) ;
#22326=CARTESIAN_POINT ( 'NONE',  ( -89.63321428752651343, -278.3514089874425963, -219.0154283612944823 ) ) ;
#22327=CARTESIAN_POINT ( 'NONE',  ( -29.83864214927978509, -273.6523845387918641, -193.7893802188771701 ) ) ;
#22328=CARTESIAN_POINT ( 'NONE',  ( 8.645876542566494294, -292.8890217288209215, -328.0101088517621974 ) ) ;
#22329=CARTESIAN_POINT ( 'NONE',  ( -11.15234293644558150, -276.1582111396244272, -201.0813940974743730 ) ) ;
#22330=CARTESIAN_POINT ( 'NONE',  ( -36.44590794135725531, -296.3033739193555789, -196.3480507826911037 ) ) ;
#22331=CARTESIAN_POINT ( 'NONE',  ( 32.73043291896075857, -295.0450869513113616, -292.2020583301730881 ) ) ;
#22332=CARTESIAN_POINT ( 'NONE',  ( 35.73365375063811200, -294.7086709965415139, -276.2107956239953523 ) ) ;
#22334=CARTESIAN_POINT ( 'NONE',  ( -110.8031928773977057, -294.7566692924618224, -254.3814173703576955 ) ) ;
#22336=CARTESIAN_POINT ( 'NONE',  ( -95.12885168234814159, -290.8613349915656840, -315.3708569196908229 ) ) ;
#22337=CARTESIAN_POINT ( 'NONE',  ( -84.48851848982423007, -296.0553699304056181, -326.1882872526021515 ) ) ;
#22338=CARTESIAN_POINT ( 'NONE',  ( -92.12060795084411779, -279.8093137243464525, -322.1822510230011858 ) ) ;
#22339=CARTESIAN_POINT ( 'NONE',  ( -109.1375609850789346, -277.5749393122844140, -243.7762220551738039 ) ) ;
#22340=CARTESIAN_POINT ( 'NONE',  ( 31.16325489794870762, -274.4502378675480259, -235.4271241777282455 ) ) ;
#22341=CARTESIAN_POINT ( 'NONE',  ( -106.5618152735892608, -282.2711395297761783, -297.8856666084632820 ) ) ;
#22342=CARTESIAN_POINT ( 'NONE',  ( -108.8483245638731489, -277.2900308443312269, -243.8793838174509574 ) ) ;
#22343=CARTESIAN_POINT ( 'NONE',  ( -70.40466981549792536, -277.6171799058535612, -202.8565369035687809 ) ) ;
#22344=CARTESIAN_POINT ( 'NONE',  ( -101.2202995325930033, -271.6247274893585768, -233.7224140011582847 ) ) ;
#22345=CARTESIAN_POINT ( 'NONE',  ( -9.296786044609506305, -276.4187681308271181, -200.7475779080155007 ) ) ;
#22347=CARTESIAN_POINT ( 'NONE',  ( -39.14647332109479549, -290.0497528034670154, -195.0147720683553700 ) ) ;
#22348=CARTESIAN_POINT ( 'NONE',  ( -40.33875888029890433, -289.0888207388034061, -347.3158505621821632 ) ) ;
#22349=CARTESIAN_POINT ( 'NONE',  ( 21.31140853968247484, -276.9069961180372843, -223.3317675410465881 ) ) ;
#22350=CARTESIAN_POINT ( 'NONE',  ( -63.70200024966509034, -295.7076995178623520, -200.2694351082888886 ) ) ;
#22351=CARTESIAN_POINT ( 'NONE',  ( -70.98628420594914701, -284.8166017956409632, -201.2800005653851372 ) ) ;
#22353=CARTESIAN_POINT ( 'NONE',  ( -49.72969589316242889, -283.8941206946745979, -196.3391989962462674 ) ) ;
#22355=CARTESIAN_POINT ( 'NONE',  ( -47.03177989159605232, -290.7212455281394341, -197.6065108542599376 ) ) ;
#22356=CARTESIAN_POINT ( 'NONE',  ( -102.0566968475360454, -283.1823730890629349, -233.8850359393497627 ) ) ;
#22359=CARTESIAN_POINT ( 'NONE',  ( 35.71804855944505874, -291.7702765558707938, -287.3667638010959422 ) ) ;
#22360=CARTESIAN_POINT ( 'NONE',  ( -93.89840380726263902, -282.3297033735481705, -321.6059562243296455 ) ) ;
#22361=CARTESIAN_POINT ( 'NONE',  ( -85.61328699062455883, -279.3328885731034461, -326.2525741948314817 ) ) ;
#22362=CARTESIAN_POINT ( 'NONE',  ( -83.05130602156704356, -286.6474361096244934, -208.8243127904968901 ) ) ;
#22363=CARTESIAN_POINT ( 'NONE',  ( -77.04906447840134831, -285.5040844853835438, -209.0449159922380602 ) ) ;
#22364=CARTESIAN_POINT ( 'NONE',  ( -21.50869651191968401, -278.2705697538941081, -342.2793170866628429 ) ) ;
#22365=CARTESIAN_POINT ( 'NONE',  ( -101.9948571213621875, -278.8895662267206603, -304.6039423004845617 ) ) ;
#22366=CARTESIAN_POINT ( 'NONE',  ( -103.6754142631424003, -287.0174945349962172, -235.2521479287557611 ) ) ;
#22369=CARTESIAN_POINT ( 'NONE',  ( -112.2738668969146829, -296.6071601269771350, -252.6362657162317191 ) ) ;
#22370=CARTESIAN_POINT ( 'NONE',  ( 32.95671788147570425, -289.8588623768545176, -295.4605049624124149 ) ) ;
#22371=CARTESIAN_POINT ( 'NONE',  ( 115.2940338803257703, -299.5541904835127980, -192.9701481807315986 ) ) ;
#22372=CARTESIAN_POINT ( 'NONE',  ( -19.11405058567862625, -282.7662352645559167, -190.3538533559490702 ) ) ;
#22373=CARTESIAN_POINT ( 'NONE',  ( -108.3753195911104399, -277.1038626329275871, -299.2698954556213380 ) ) ;
#22375=CARTESIAN_POINT ( 'NONE',  ( 6.140605363105556158, -292.8731093898400673, -333.0011896450453719 ) ) ;
#22376=CARTESIAN_POINT ( 'NONE',  ( 17.39272361777657139, -288.3721519867979168, -220.9980796664841591 ) ) ;
#22377=CARTESIAN_POINT ( 'NONE',  ( -109.8848725510550537, -280.5041089334150115, -255.6187524875688837 ) ) ;
#22378=CARTESIAN_POINT ( 'NONE',  ( 21.05056746609663421, -289.6464695405196608, -319.6454905534583304 ) ) ;
#22379=CARTESIAN_POINT ( 'NONE',  ( -112.0869438188197904, -286.4730103280032267, -276.5376212275803027 ) ) ;
#22380=CARTESIAN_POINT ( 'NONE',  ( -112.9965772427299129, -278.8989257709359890, -255.9609180133413133 ) ) ;
#22382=CARTESIAN_POINT ( 'NONE',  ( -37.80804921678049624, -296.0663921191614349, -195.7177704858326308 ) ) ;
#22383=CARTESIAN_POINT ( 'NONE',  ( 36.91470676653590743, -291.4538943213717630, -256.3861319210874399 ) ) ;
#22384=CARTESIAN_POINT ( 'NONE',  ( -84.56525879359641351, -279.2556363533514059, -209.4747704247852766 ) ) ;
#22385=CARTESIAN_POINT ( 'NONE',  ( -24.40406663599654280, -276.0793243424434422, -197.2095273029512725 ) ) ;
#22387=CARTESIAN_POINT ( 'NONE',  ( 21.31550574532285580, -296.6948066931273615, -317.0979686699210447 ) ) ;
#22388=CARTESIAN_POINT ( 'NONE',  ( -60.54014508124423344, -271.9953094507193896, -197.9473554753666633 ) ) ;
#22390=CARTESIAN_POINT ( 'NONE',  ( -51.83343822743881901, -279.3694759279116511, -198.6994432783881450 ) ) ;
#22391=CARTESIAN_POINT ( 'NONE',  ( 33.82111179947592916, -277.1203923759173904, -298.8566777769632381 ) ) ;
#22392=CARTESIAN_POINT ( 'NONE',  ( -77.85136105650438765, -298.9218706697556058, -208.8641990159432282 ) ) ;
#22393=CARTESIAN_POINT ( 'NONE',  ( -104.2179396335195207, -283.1191518854671472, -308.1568553186463078 ) ) ;
#22394=CARTESIAN_POINT ( 'NONE',  ( -48.18763493631013972, -290.9520428080189163, -343.6271877368289438 ) ) ;
#22395=CARTESIAN_POINT ( 'NONE',  ( -105.8989597768701572, -298.5064153037426991, -236.8557467664184060 ) ) ;
#22396=CARTESIAN_POINT ( 'NONE',  ( -109.4821066213579286, -298.0841180943501172, -244.5973746796761077 ) ) ;
#22397=CARTESIAN_POINT ( 'NONE',  ( 30.05655093047798587, -295.9829947587128913, -302.9999946361118646 ) ) ;
#22398=CARTESIAN_POINT ( 'NONE',  ( -15.62417824309960857, -280.7703005196200934, -341.9738100654732307 ) ) ;
#22399=CARTESIAN_POINT ( 'NONE',  ( -43.59533959331694319, -271.9929972876396391, -195.9268828857573226 ) ) ;
#22400=CARTESIAN_POINT ( 'NONE',  ( -70.73422973412071713, -287.2191737242491172, -201.8674731295454876 ) ) ;
#22401=CARTESIAN_POINT ( 'NONE',  ( -26.44245367431672378, -287.8306597628556460, -342.9067445073270619 ) ) ;
#22402=CARTESIAN_POINT ( 'NONE',  ( 140.3257785139489044, 179.6804926070224155, -241.2945171362309225 ) ) ;
#22404=CARTESIAN_POINT ( 'NONE',  ( -74.15945537472130411, -288.1062803915087898, -337.3317089384698306 ) ) ;
#22405=CARTESIAN_POINT ( 'NONE',  ( 21.18788884857454136, -287.8315694605126396, -314.0440985156255351 ) ) ;
#22406=ORIENTED_EDGE ( 'NONE', *, *, #43878, .F. ) ;
#22407=CARTESIAN_POINT ( 'NONE',  ( -93.70195066783594484, -286.3434533262437753, -218.2735178149416697 ) ) ;
#22408=CARTESIAN_POINT ( 'NONE',  ( 9.680902497258630390, -276.7170976854366700, -326.2266917200656167 ) ) ;
#22409=CARTESIAN_POINT ( 'NONE',  ( 38.54807015514720803, -292.3291765352909692, -258.9483610207844322 ) ) ;
#22410=CARTESIAN_POINT ( 'NONE',  ( -99.70094065985946941, -284.6051363360588766, -315.4460690264696154 ) ) ;
#22412=CARTESIAN_POINT ( 'NONE',  ( 38.71905078978815595, -282.9950219252702368, -264.2398500435169240 ) ) ;
#22413=CARTESIAN_POINT ( 'NONE',  ( -0.3818607462137903474, -282.9078857694941007, -337.9017119002714367 ) ) ;
#22414=CARTESIAN_POINT ( 'NONE',  ( -32.96598651701893345, -280.4420792808553529, -197.4711967505822372 ) ) ;
#22415=CARTESIAN_POINT ( 'NONE',  ( -70.86830917777322725, -196.3883269678753152, -360.5550801755780981 ) ) ;
#22416=CARTESIAN_POINT ( 'NONE',  ( -109.5836222876633315, -280.3007506750664675, -289.8837487389042735 ) ) ;
#22417=CARTESIAN_POINT ( 'NONE',  ( 160.1180839598566195, 220.5390337495420283, -204.7865604871097105 ) ) ;
#22418=CARTESIAN_POINT ( 'NONE',  ( 178.1438528349047203, 252.3106890361019907, -164.5180092551200630 ) ) ;
#22419=CARTESIAN_POINT ( 'NONE',  ( -93.03006199293928091, -272.4229359308798166, -222.8927779124822450 ) ) ;
#22420=CARTESIAN_POINT ( 'NONE',  ( -13.80683339856973824, -294.2623488004030037, -343.6116261796562981 ) ) ;
#22421=CARTESIAN_POINT ( 'NONE',  ( 103.8198587862023459, 114.2352195572753573, -279.7816234916556937 ) ) ;
#22422=CARTESIAN_POINT ( 'NONE',  ( -106.3909035283975868, -271.6620883614435797, -237.4141032285587869 ) ) ;
#22423=CARTESIAN_POINT ( 'NONE',  ( -108.5026076409199334, -288.6941695497823162, -290.1089206472752835 ) ) ;
#22424=CARTESIAN_POINT ( 'NONE',  ( -97.39390445610423797, -297.8116808824607915, -314.0245089040078597 ) ) ;
#22425=CARTESIAN_POINT ( 'NONE',  ( 36.17319654799493378, -288.8400893544101109, -268.2819100810057762 ) ) ;
#22427=CARTESIAN_POINT ( 'NONE',  ( -97.21635824852825181, -296.8475193097922897, -318.4219584456608345 ) ) ;
#22428=CARTESIAN_POINT ( 'NONE',  ( 20.38542466001556619, -287.4142440313824522, -225.5775550876500972 ) ) ;
#22429=CARTESIAN_POINT ( 'NONE',  ( -63.43893346195628169, -272.6402136818743998, -198.2471323640708363 ) ) ;
#22430=CARTESIAN_POINT ( 'NONE',  ( 19.41732322056124005, -295.0612952465291414, -322.2321828044285894 ) ) ;
#22431=CARTESIAN_POINT ( 'NONE',  ( -3.354190619114073346, -292.9812325736764933, -201.3221324680027919 ) ) ;
#22432=CARTESIAN_POINT ( 'NONE',  ( -103.5572096936009530, -291.1336785839383765, -239.6282968061431120 ) ) ;
#22434=CARTESIAN_POINT ( 'NONE',  ( -105.5539529197887703, -274.8968957535345794, -237.8587678488131303 ) ) ;
#22435=CARTESIAN_POINT ( 'NONE',  ( 1.009986396717812207, -273.3470126578176291, -204.0348487712289511 ) ) ;
#22437=CARTESIAN_POINT ( 'NONE',  ( -104.7366608798621144, -278.5409080611475474, -233.2471560768232166 ) ) ;
#22438=CARTESIAN_POINT ( 'NONE',  ( -6.172774650221306558, -272.8685870005797938, -203.4661368404431983 ) ) ;
#22439=CARTESIAN_POINT ( 'NONE',  ( -96.53908632886891894, -274.2357801045013730, -227.0344700584482212 ) ) ;
#22440=CARTESIAN_POINT ( 'NONE',  ( 26.83696552098341570, -276.0118057899703672, -234.9778805313569308 ) ) ;
#22441=CARTESIAN_POINT ( 'NONE',  ( -3.868772761384751124, -300.0647303613785652, -194.1521717235641518 ) ) ;
#22442=CARTESIAN_POINT ( 'NONE',  ( -4.729988934791962585, -274.6448911267726771, -338.3082351913516277 ) ) ;
#22443=CARTESIAN_POINT ( 'NONE',  ( -72.16584159823331390, -296.1770615841671770, -334.6495987859615866 ) ) ;
#22444=CARTESIAN_POINT ( 'NONE',  ( 19.27489436450392901, -292.7883262167277962, -317.3710759365084755 ) ) ;
#22446=CARTESIAN_POINT ( 'NONE',  ( -70.26898557065474904, -277.9668062097417760, -339.9120142852159461 ) ) ;
#22447=CARTESIAN_POINT ( 'NONE',  ( 23.05113954428155765, -275.1482639459219399, -229.3301015376934799 ) ) ;
#22449=CARTESIAN_POINT ( 'NONE',  ( -104.9881786169803206, -283.7026935975775928, -234.5090665878209393 ) ) ;
#22450=CARTESIAN_POINT ( 'NONE',  ( -102.9890394261793602, -298.0648251094286252, -307.0796874485572516 ) ) ;
#22452=CARTESIAN_POINT ( 'NONE',  ( -81.56808382118443035, -284.6296206617756184, -212.0805147610245456 ) ) ;
#22453=CARTESIAN_POINT ( 'NONE',  ( -109.2692225733536588, -277.0190558710642676, -252.9138966800696835 ) ) ;
#22454=CARTESIAN_POINT ( 'NONE',  ( -76.68606469585640184, -276.1643811171157381, -332.6094468953904197 ) ) ;
#22455=CARTESIAN_POINT ( 'NONE',  ( -110.8647083862474574, -286.3613181809882349, -285.2360512963271049 ) ) ;
#22456=CARTESIAN_POINT ( 'NONE',  ( -2.739948351401155335, -275.7255210193334847, -205.6320728821359580 ) ) ;
#22458=CARTESIAN_POINT ( 'NONE',  ( 38.90666704328149450, -273.9624179993852522, -271.1835598520960389 ) ) ;
#22459=CARTESIAN_POINT ( 'NONE',  ( -69.20887382580913538, -281.6341555470060598, -202.2698216998622058 ) ) ;
#22461=CARTESIAN_POINT ( 'NONE',  ( -49.14437751031390178, -287.8231763335015216, -195.6758789415342790 ) ) ;
#22464=CARTESIAN_POINT ( 'NONE',  ( 20.78113675958304896, -290.8987050903985505, -222.9414242994105564 ) ) ;
#22465=CARTESIAN_POINT ( 'NONE',  ( 82.16127410785169616, -298.5792860220823854, -197.1167434283082969 ) ) ;
#22466=CARTESIAN_POINT ( 'NONE',  ( -73.02658463023458069, -296.3628394684810701, -206.2228336009708300 ) ) ;
#22467=CARTESIAN_POINT ( 'NONE',  ( -95.23962990857572208, -289.3376935585451974, -223.8791649500989536 ) ) ;
#22468=CARTESIAN_POINT ( 'NONE',  ( -84.42323508662160236, -232.9070939334762329, -346.4289530206739300 ) ) ;
#22469=CARTESIAN_POINT ( 'NONE',  ( -61.12666982825986395, -295.7433451171331171, -199.1776039324604142 ) ) ;
#22470=CARTESIAN_POINT ( 'NONE',  ( -103.2098144371225317, -288.5249129832526478, -308.9896842094865406 ) ) ;
#22471=CARTESIAN_POINT ( 'NONE',  ( 10.44202075880268943, -283.9800635391399624, -326.6702840655408409 ) ) ;
#22472=CARTESIAN_POINT ( 'NONE',  ( -110.1436449404158964, -282.5146899080751837, -292.1744620578613194 ) ) ;
#22473=CARTESIAN_POINT ( 'NONE',  ( -4.548414203436010439, -284.0365622864845818, -336.2396070149167144 ) ) ;
#22474=CARTESIAN_POINT ( 'NONE',  ( -67.84238802978804017, -284.2658978095436169, -336.8615673419376435 ) ) ;
#22476=CARTESIAN_POINT ( 'NONE',  ( -105.0248430746607511, -292.0959797869946328, -303.6066591384906701 ) ) ;
#22477=CARTESIAN_POINT ( 'NONE',  ( -18.55924196096452050, -274.6208300385341659, -195.6538195044522581 ) ) ;
#22478=CARTESIAN_POINT ( 'NONE',  ( -54.20449545069922692, -287.3467715438604273, -344.0691402898726210 ) ) ;
#22479=CARTESIAN_POINT ( 'NONE',  ( 38.92417607413189273, -275.4194924690856965, -259.7537560528111271 ) ) ;
#22480=CARTESIAN_POINT ( 'NONE',  ( 9.274592697482173520, -296.3884727372923749, -328.7265195592930240 ) ) ;
#22482=CARTESIAN_POINT ( 'NONE',  ( 99.44099354567467230, -302.2645883696979467, -195.3030568020281521 ) ) ;
#22483=CARTESIAN_POINT ( 'NONE',  ( -45.71215689695105766, -281.8451461596557124, -343.4273801591559732 ) ) ;
#22484=CARTESIAN_POINT ( 'NONE',  ( -111.4948372707474675, -276.3943856883842045, -282.6631779616280937 ) ) ;
#22486=CARTESIAN_POINT ( 'NONE',  ( -31.95916909530536998, -296.5183538027648638, -194.1625494488639561 ) ) ;
#22487=CARTESIAN_POINT ( 'NONE',  ( 33.61011650764340430, -274.6688226728804807, -252.7619025280739606 ) ) ;
#22488=CARTESIAN_POINT ( 'NONE',  ( -25.31482904837751136, -293.7282247890242388, -197.6038423582666894 ) ) ;
#22489=CARTESIAN_POINT ( 'NONE',  ( 19.88511512992895192, -295.1370610797394534, -316.0812238694236953 ) ) ;
#22490=CARTESIAN_POINT ( 'NONE',  ( -90.40478407308286535, -287.0488278596349687, -218.6902306258596127 ) ) ;
#22491=CARTESIAN_POINT ( 'NONE',  ( 37.49718685151719200, -295.1717421387989475, -285.7801740642635764 ) ) ;
#22492=CARTESIAN_POINT ( 'NONE',  ( 26.11215191008017200, -295.4340730176405714, -313.1034498590222483 ) ) ;
#22493=CARTESIAN_POINT ( 'NONE',  ( -110.2121603534482119, -296.4428146462902305, -266.0141614575670133 ) ) ;
#22494=CARTESIAN_POINT ( 'NONE',  ( -102.0160429505700677, -292.0435366280884182, -308.4400537465915022 ) ) ;
#22495=CARTESIAN_POINT ( 'NONE',  ( -81.55982012790093449, -283.8019995466293039, -333.4637324805561889 ) ) ;
#22496=CARTESIAN_POINT ( 'NONE',  ( -96.82829257484100083, -271.3295856147320251, -223.4393660561182458 ) ) ;
#22497=CARTESIAN_POINT ( 'NONE',  ( -18.17997500119582455, -286.1256957482785310, -195.7283489597987227 ) ) ;
#22498=CARTESIAN_POINT ( 'NONE',  ( -62.31692380987604452, -279.3583674818408440, -340.7586879571641703 ) ) ;
#22500=CARTESIAN_POINT ( 'NONE',  ( -38.61649543187973421, -284.8307717300806985, -196.9625654323137098 ) ) ;
#22502=CARTESIAN_POINT ( 'NONE',  ( 21.69691511056095123, -286.1869833321935630, -316.6358973213487502 ) ) ;
#22503=CARTESIAN_POINT ( 'NONE',  ( -103.7001496316577516, -277.1730595717525603, -233.7979991656895606 ) ) ;
#22504=CARTESIAN_POINT ( 'NONE',  ( -108.4555765497910471, -262.4588243622614527, -317.8183916042563055 ) ) ;
#22505=CARTESIAN_POINT ( 'NONE',  ( -65.11080558841855748, -285.1870441594747945, -202.7286816938384959 ) ) ;
#22506=CARTESIAN_POINT ( 'NONE',  ( 35.23783331925652362, -283.0692704806687061, -295.0254507566252187 ) ) ;
#22507=CARTESIAN_POINT ( 'NONE',  ( -73.07500556531870473, -288.5727144053486199, -338.3166214257569209 ) ) ;
#22508=CARTESIAN_POINT ( 'NONE',  ( -39.91530906589232330, -278.6840701793875041, -346.5305779452963293 ) ) ;
#22509=CARTESIAN_POINT ( 'NONE',  ( -86.76377785003018062, -279.0376679027629052, -328.8321039229232383 ) ) ;
#22510=CARTESIAN_POINT ( 'NONE',  ( -43.74897457045302218, -279.8023882867135512, -197.5926137027811649 ) ) ;
#22511=CARTESIAN_POINT ( 'NONE',  ( -32.61143097120459089, -276.0919350915609698, -195.8535353109436983 ) ) ;
#22512=CARTESIAN_POINT ( 'NONE',  ( 38.07058928899563455, -293.7467003975645525, -285.9170366270830641 ) ) ;
#22513=CARTESIAN_POINT ( 'NONE',  ( -85.77091236000565289, -287.7461447193713866, -327.2312823814820604 ) ) ;
#22514=CARTESIAN_POINT ( 'NONE',  ( -105.2999646326113918, -292.6020122703067159, -235.7756756215604526 ) ) ;
#22515=CARTESIAN_POINT ( 'NONE',  ( 33.41143883832940276, -292.7254602204116054, -289.5978569015352377 ) ) ;
#22516=CARTESIAN_POINT ( 'NONE',  ( 28.41174480821354820, -293.6499285505595935, -302.2357345633083128 ) ) ;
#22517=CARTESIAN_POINT ( 'NONE',  ( -112.3405887715641143, -291.8337275631249668, -254.2785198051710722 ) ) ;
#22518=CARTESIAN_POINT ( 'NONE',  ( 34.58723590186753682, -282.3763117907469109, -283.4743403701189095 ) ) ;
#22519=CARTESIAN_POINT ( 'NONE',  ( -89.99273195207298670, -272.3891525716839510, -214.4254113431359485 ) ) ;
#22520=CARTESIAN_POINT ( 'NONE',  ( -68.00559948550848333, -290.0957112385090682, -340.8808887071532467 ) ) ;
#22521=CARTESIAN_POINT ( 'NONE',  ( -95.34029919066875891, -282.0244653891793973, -319.1302302714141774 ) ) ;
#22522=CARTESIAN_POINT ( 'NONE',  ( -65.43535045956707563, -289.7426903436191310, -342.0867616799149005 ) ) ;
#22523=CARTESIAN_POINT ( 'NONE',  ( 11.14492882572142030, -287.0787179588227787, -215.6934204259425485 ) ) ;
#22524=CARTESIAN_POINT ( 'NONE',  ( 82.64890176555634582, -299.5541904835127980, -195.3611179825600175 ) ) ;
#22525=CARTESIAN_POINT ( 'NONE',  ( 178.0079900246404350, 253.3980089039855557, -165.2740606419443736 ) ) ;
#22526=CARTESIAN_POINT ( 'NONE',  ( 153.0936500521454775, 204.7395457004011234, -214.2756457972470230 ) ) ;
#22527=CARTESIAN_POINT ( 'NONE',  ( -62.35456707728842218, -278.9155811341140634, -201.5547681482764517 ) ) ;
#22528=CARTESIAN_POINT ( 'NONE',  ( -27.50333598972031979, -279.1002600405496992, -197.6637688007097040 ) ) ;
#22529=CARTESIAN_POINT ( 'NONE',  ( 20.02295116130064301, -274.5217958678194918, -218.9501269829323746 ) ) ;
#22530=CARTESIAN_POINT ( 'NONE',  ( -68.78722892216374873, -196.9352846320093136, -357.8051255537320685 ) ) ;
#22531=CARTESIAN_POINT ( 'NONE',  ( -112.4138460204593599, -277.3072307530179614, -256.0511723597472269 ) ) ;
#22532=CARTESIAN_POINT ( 'NONE',  ( -7.867465775643090353, -280.6841339257362051, -338.9403882776479691 ) ) ;
#22533=CARTESIAN_POINT ( 'NONE',  ( -25.04935531457887876, -296.6577441006658660, -345.4002883162921194 ) ) ;
#22534=CARTESIAN_POINT ( 'NONE',  ( -62.82806531799420213, -292.2035393942699102, -201.8889803566277408 ) ) ;
#22535=CARTESIAN_POINT ( 'NONE',  ( -89.01965424845269581, -288.4823313306475825, -322.6165725824428137 ) ) ;
#22536=CARTESIAN_POINT ( 'NONE',  ( 19.32610810018613989, -299.2361782822673604, -193.4180472008978597 ) ) ;
#22537=CARTESIAN_POINT ( 'NONE',  ( -110.0990318594879511, -296.6325513537497613, -276.9017552651960159 ) ) ;
#22540=CARTESIAN_POINT ( 'NONE',  ( -111.6450297054304315, -280.2964986378397043, -284.1553986849187368 ) ) ;
#22541=CARTESIAN_POINT ( 'NONE',  ( 18.18972221567073078, -281.9528689193521132, -222.4828179980798950 ) ) ;
#22542=CARTESIAN_POINT ( 'NONE',  ( -97.11769008258531244, -279.6767489313735382, -317.2738565767593286 ) ) ;
#22543=CARTESIAN_POINT ( 'NONE',  ( 33.87615759099319490, -280.8360735141135933, -287.4856144781021499 ) ) ;
#22544=CARTESIAN_POINT ( 'NONE',  ( -43.52114399251894383, -272.4526933469902588, -196.8761311456931651 ) ) ;
#22547=CARTESIAN_POINT ( 'NONE',  ( 24.24437521223253711, -276.9675000215099772, -316.3101565485692959 ) ) ;
#22548=CARTESIAN_POINT ( 'NONE',  ( 25.97444438457528193, -278.0943193268141158, -310.6580346857036261 ) ) ;
#22549=CARTESIAN_POINT ( 'NONE',  ( -88.82857463648720397, -276.3334075857380299, -326.8209093824336264 ) ) ;
#22552=CARTESIAN_POINT ( 'NONE',  ( 20.36700430224048830, -284.1986966210026253, -318.8184418773226980 ) ) ;
#22553=CARTESIAN_POINT ( 'NONE',  ( -99.84426448602748394, -290.2718940567323216, -232.3344013821432270 ) ) ;
#22554=CARTESIAN_POINT ( 'NONE',  ( 18.28350567566745966, -286.1730485862634623, -217.1886532087675050 ) ) ;
#22555=CARTESIAN_POINT ( 'NONE',  ( -21.18859054937971464, -281.0820905885889260, -342.6430061844567376 ) ) ;
#22556=CARTESIAN_POINT ( 'NONE',  ( -87.34239674746299897, -282.3401877989085165, -324.4244157405486249 ) ) ;
#22558=CARTESIAN_POINT ( 'NONE',  ( -11.61828678393587566, -281.5997044746429196, -201.5655645842719252 ) ) ;
#22560=CARTESIAN_POINT ( 'NONE',  ( -94.74563448016067468, -282.2672103572789410, -320.4732795560731802 ) ) ;
#22561=CARTESIAN_POINT ( 'NONE',  ( -112.2349716561223261, -298.4897306966552151, -275.2354500860950566 ) ) ;
#22562=CARTESIAN_POINT ( 'NONE',  ( -106.6713477330333575, -279.8078359778444906, -246.6085214829126642 ) ) ;
#22563=CARTESIAN_POINT ( 'NONE',  ( -109.1815857544270330, -286.8388378424853045, -248.0710490295336683 ) ) ;
#22564=DIRECTION ( 'NONE',  ( 0.000000000000000000, 0.000000000000000000, -1.000000000000000000 ) ) ;
#22566=CARTESIAN_POINT ( 'NONE',  ( 38.27060701774458096, -295.4713574460122913, -270.2865095391824184 ) ) ;
#22567=CARTESIAN_POINT ( 'NONE',  ( 10.93243487874202735, -274.3840315797502853, -327.7597985865685928 ) ) ;
#22568=CARTESIAN_POINT ( 'NONE',  ( -67.99886345592852877, -288.6417004884300468, -340.8188865930616771 ) ) ;
#22569=CARTESIAN_POINT ( 'NONE',  ( 34.08759011211144241, -291.7097103146563768, -251.8058784879941356 ) ) ;
#22570=CARTESIAN_POINT ( 'NONE',  ( -95.67459479516085707, -276.6122773088797544, -315.0658926624392961 ) ) ;
#22571=CARTESIAN_POINT ( 'NONE',  ( -111.0335929686983860, -294.5700828966379845, -279.7387666122154997 ) ) ;
#22572=CARTESIAN_POINT ( 'NONE',  ( -70.45782826173180524, -292.9212209856526101, -204.7519300827885900 ) ) ;
#22573=CARTESIAN_POINT ( 'NONE',  ( -85.28047601435906699, -280.1948066931273615, -330.5268031993605859 ) ) ;
#22574=CARTESIAN_POINT ( 'NONE',  ( -44.74777653480868622, -293.6240174303553090, -346.3604583207958285 ) ) ;
#22575=CARTESIAN_POINT ( 'NONE',  ( 29.52630890934421259, -288.7351815748234003, -239.1343701470424605 ) ) ;
#22576=CARTESIAN_POINT ( 'NONE',  ( -111.6443060708512292, -288.9943751328019061, -254.3908009182405578 ) ) ;
#22577=CARTESIAN_POINT ( 'NONE',  ( -29.08916763974091424, -290.3707935216937130, -343.4861521648430767 ) ) ;
#22578=CYLINDRICAL_SURFACE ( 'NONE', #71327, 1.897123461337413275 ) ;
#22579=CARTESIAN_POINT ( 'NONE',  ( -88.76732337151497632, -290.5999965870382198, -322.3996325732541663 ) ) ;
#22581=CARTESIAN_POINT ( 'NONE',  ( 82.70991478241074901, -294.7622393454342955, -197.7570935515998087 ) ) ;
#22582=CARTESIAN_POINT ( 'NONE',  ( 5.348826291215152295, -289.6933149964566496, -333.9655806547092425 ) ) ;
#22583=CARTESIAN_POINT ( 'NONE',  ( -106.9827673550305320, -276.9461017368034845, -241.5769460174636265 ) ) ;
#22584=CARTESIAN_POINT ( 'NONE',  ( -36.75697793451085005, -280.3925927418611082, -193.3714407658291350 ) ) ;
#22585=CARTESIAN_POINT ( 'NONE',  ( -10.71333275034624499, -282.3810366851079152, -342.6442961314813829 ) ) ;
#22586=CARTESIAN_POINT ( 'NONE',  ( 27.41025551473672550, -286.0588070559125526, -308.3079504644597932 ) ) ;
#22587=DIRECTION ( 'NONE',  ( -1.000000000000000000, -0.000000000000000000, -0.000000000000000000 ) ) ;
#22588=CARTESIAN_POINT ( 'NONE',  ( 1.058847993968061063, -278.7097230569691533, -206.7700097325325999 ) ) ;
#22589=CARTESIAN_POINT ( 'NONE',  ( -30.42535961952033929, -280.9644985858746509, -345.0415363157139268 ) ) ;
#22590=CARTESIAN_POINT ( 'NONE',  ( 181.0082777314984241, 252.6787652719002040, -164.6486270092325128 ) ) ;
#22591=CARTESIAN_POINT ( 'NONE',  ( -98.85734849419212367, -277.6373887186409206, -225.1889591390722956 ) ) ;
#22592=CARTESIAN_POINT ( 'NONE',  ( -95.11098289941921280, -282.7875832412171917, -320.8012059922886579 ) ) ;
#22593=CARTESIAN_POINT ( 'NONE',  ( 52.01832293716342548, -300.1390605925521982, -197.1111399590675148 ) ) ;
#22594=CARTESIAN_POINT ( 'NONE',  ( -87.66208520482945232, -274.7911321845207340, -212.7888858945432276 ) ) ;
#22595=CARTESIAN_POINT ( 'NONE',  ( -16.37885764104276021, -276.4404811782455909, -340.3615981858769146 ) ) ;
#22596=CARTESIAN_POINT ( 'NONE',  ( -79.04113971308001396, -297.6142186600198443, -332.7628848608052863 ) ) ;
#22597=CARTESIAN_POINT ( 'NONE',  ( -105.1549656640309109, -290.2472513649459529, -306.8352323904114769 ) ) ;
#22598=CARTESIAN_POINT ( 'NONE',  ( 35.60141979152266600, -279.3798612572268212, -250.5986592957176811 ) ) ;
#22599=CARTESIAN_POINT ( 'NONE',  ( 23.10939165632237291, -292.7473551402242720, -222.6465942237843478 ) ) ;
#22601=CARTESIAN_POINT ( 'NONE',  ( -31.86568611225878911, -288.0402444912931514, -343.4421837259578183 ) ) ;
#22602=CARTESIAN_POINT ( 'NONE',  ( 36.83465199597038975, -291.6943164942666158, -281.4457665902666008 ) ) ;
#22605=CARTESIAN_POINT ( 'NONE',  ( -88.70878431863918934, -289.3050255424132047, -322.3169752399836625 ) ) ;
#22607=CARTESIAN_POINT ( 'NONE',  ( -7.445859927967695135, -287.3757928195747127, -199.6006166529968198 ) ) ;
#22608=CARTESIAN_POINT ( 'NONE',  ( -6.941161984400275209, -297.1233781216987495, -333.4151289067050357 ) ) ;
#22609=CARTESIAN_POINT ( 'NONE',  ( 22.09681380320278876, -293.2652029048347231, -318.9603791118698268 ) ) ;
#22610=CARTESIAN_POINT ( 'NONE',  ( 17.48464388436363848, -283.6042872458888269, -323.7975903708006058 ) ) ;
#22611=CARTESIAN_POINT ( 'NONE',  ( -110.3188846175833362, -284.3422696491132911, -273.6360186376242041 ) ) ;
#22612=CARTESIAN_POINT ( 'NONE',  ( 22.87949496039619746, -277.4518885941686790, -312.5751226865164654 ) ) ;
#22613=CARTESIAN_POINT ( 'NONE',  ( 24.27681434211216072, -292.1466705259947503, -312.5822780444832460 ) ) ;
#22614=CARTESIAN_POINT ( 'NONE',  ( 25.62432395733213752, -273.8299538586905442, -232.5477868144641604 ) ) ;
#22616=CARTESIAN_POINT ( 'NONE',  ( -32.04911714649202992, -124.5213432794980974, -365.6788127701597659 ) ) ;
#22617=CARTESIAN_POINT ( 'NONE',  ( 29.55419283905159489, -293.7148451698776057, -308.5566313757004764 ) ) ;
#22618=CARTESIAN_POINT ( 'NONE',  ( -10.24820624270802050, -288.3286735793968205, -201.0129434889128390 ) ) ;
#22619=CARTESIAN_POINT ( 'NONE',  ( -101.3626108634006187, -297.0732757896138878, -312.6805340037668088 ) ) ;
#22621=CARTESIAN_POINT ( 'NONE',  ( -52.11763068027443779, -286.5093794383482191, -198.7680698273709083 ) ) ;
#22622=CARTESIAN_POINT ( 'NONE',  ( -107.2000071094652611, -278.0203483367379249, -238.4112205248872840 ) ) ;
#22623=CARTESIAN_POINT ( 'NONE',  ( -77.02251135453006725, -296.2201432068360987, -336.2922210778831413 ) ) ;
#22624=CARTESIAN_POINT ( 'NONE',  ( -62.37820261873216765, -287.5138601287436018, -341.9251985713036106 ) ) ;
#22626=CARTESIAN_POINT ( 'NONE',  ( 39.21651000224836991, -293.9921059565856467, -278.8883081489851747 ) ) ;
#22627=CARTESIAN_POINT ( 'NONE',  ( -107.4167836424392277, -291.1575248568599932, -249.7845368836059947 ) ) ;
#22630=CARTESIAN_POINT ( 'NONE',  ( -38.36988802030046486, -140.4513536129776412, -361.1260187711050662 ) ) ;
#22632=CARTESIAN_POINT ( 'NONE',  ( 37.99366567511329151, -289.2294910628455114, -282.8191850300649435 ) ) ;
#22633=CARTESIAN_POINT ( 'NONE',  ( 13.84574458161073807, -284.1952119285919025, -206.2264541496106460 ) ) ;
#22634=ORIENTED_EDGE ( 'NONE', *, *, #3118, .F. ) ;
#22635=CARTESIAN_POINT ( 'NONE',  ( -113.9415690105022065, -277.9927306780792264, -263.0154000966647345 ) ) ;
#22636=CARTESIAN_POINT ( 'NONE',  ( 34.87631109955725606, -283.2990262893106319, -250.7012581078978428 ) ) ;
#22637=CARTESIAN_POINT ( 'NONE',  ( -10.86276471313879632, -92.93242878793211048, -358.8789665578360086 ) ) ;
#22638=CARTESIAN_POINT ( 'NONE',  ( -106.4802662602394463, -282.7069542370766158, -302.8951765131579350 ) ) ;
#22639=CARTESIAN_POINT ( 'NONE',  ( -18.12489030421997427, -286.8825176474620093, -342.3315523510055414 ) ) ;
#22640=CARTESIAN_POINT ( 'NONE',  ( -27.18592835138849040, -276.0401994777554933, -195.2274848994934757 ) ) ;
#22641=CARTESIAN_POINT ( 'NONE',  ( -68.07912563937648542, -298.1297021990621374, -204.0662291882327395 ) ) ;
#22642=CARTESIAN_POINT ( 'NONE',  ( 6.342712854686643809, -293.1299441708004565, -329.5254223798096405 ) ) ;
#22643=CARTESIAN_POINT ( 'NONE',  ( 26.19170978608781297, -281.6303565386378978, -226.9459562399169670 ) ) ;
#22644=CARTESIAN_POINT ( 'NONE',  ( -13.78539871757494240, -276.7378892667989589, -339.5091228563138088 ) ) ;
#22645=CARTESIAN_POINT ( 'NONE',  ( -108.7044529258909336, -278.1102324348433399, -254.4529716086750852 ) ) ;
#22646=CARTESIAN_POINT ( 'NONE',  ( -64.80229165145864556, -274.7814801134947515, -198.7410636321780544 ) ) ;
#22647=CARTESIAN_POINT ( 'NONE',  ( -37.14163223813358883, -275.9700018962540184, -347.0647523795010443 ) ) ;
#22649=CARTESIAN_POINT ( 'NONE',  ( -67.38406429639361761, -275.4459653811994713, -339.0949792678342192 ) ) ;
#22650=CARTESIAN_POINT ( 'NONE',  ( -95.12393327783939867, -297.2967488081391139, -320.3593162127646679 ) ) ;
#22653=CARTESIAN_POINT ( 'NONE',  ( 4.892272440320851068, -287.7171646901823010, -210.3780776303739231 ) ) ;
#22654=CARTESIAN_POINT ( 'NONE',  ( -110.1307546509781048, -286.0344040821171347, -292.2174348960887187 ) ) ;
#22655=CARTESIAN_POINT ( 'NONE',  ( 18.74529896702300036, -286.2360095918974139, -223.4572749630345356 ) ) ;
#22656=CARTESIAN_POINT ( 'NONE',  ( -97.55004068307407294, -276.3623267449929131, -313.0608915440399755 ) ) ;
#22657=CARTESIAN_POINT ( 'NONE',  ( -108.9464186807513073, -286.1575422643813340, -289.9955221357749338 ) ) ;
#22658=CARTESIAN_POINT ( 'NONE',  ( -110.6537889255837968, -277.1362267581268952, -262.3869392697350804 ) ) ;
#22659=CARTESIAN_POINT ( 'NONE',  ( -61.88039495705736925, -278.4582917975523628, -339.4953147396041118 ) ) ;
#22661=CARTESIAN_POINT ( 'NONE',  ( 35.64808926029486713, -275.9887229816575882, -266.1291621752004062 ) ) ;
#22662=CARTESIAN_POINT ( 'NONE',  ( -7.608933189270027597, -281.2349225782449480, -199.4940308079887643 ) ) ;
#22663=CARTESIAN_POINT ( 'NONE',  ( 39.46816469795334115, -282.1107011621401739, -275.6504160986082752 ) ) ;
#22667=CARTESIAN_POINT ( 'NONE',  ( -71.33076387494281789, -291.3565721278113756, -338.0741080922221613 ) ) ;
#22668=CARTESIAN_POINT ( 'NONE',  ( -95.09709677030082275, -288.5544328190668466, -320.5369331965659399 ) ) ;
#22670=CARTESIAN_POINT ( 'NONE',  ( -107.7610049202036038, -295.4875981973454486, -290.2035785117758451 ) ) ;
#22671=CARTESIAN_POINT ( 'NONE',  ( -8.541687487851248761, -291.7679564255004721, -199.0598412858064705 ) ) ;
#22672=CARTESIAN_POINT ( 'NONE',  ( 32.04577529113598899, -286.3594122793471684, -295.1821978675232003 ) ) ;
#22673=CARTESIAN_POINT ( 'NONE',  ( -17.13470088807447667, -290.5563125151219879, -199.1063071835174298 ) ) ;
#22674=CARTESIAN_POINT ( 'NONE',  ( 29.16330360798184884, -288.3401925010050491, -239.3093067361381543 ) ) ;
#22675=CARTESIAN_POINT ( 'NONE',  ( -37.30987171927208124, -291.5519495502701943, -345.3611179825600175 ) ) ;
#22676=CARTESIAN_POINT ( 'NONE',  ( 25.77581920227296663, -290.0990160658569152, -310.9683981270106301 ) ) ;
#22677=CARTESIAN_POINT ( 'NONE',  ( -7.667696378681542413, -286.6639937676915224, -339.4364524732916948 ) ) ;
#22678=CARTESIAN_POINT ( 'NONE',  ( -73.90389798382059894, -284.4914329886111091, -333.8745104777723895 ) ) ;
#22679=CARTESIAN_POINT ( 'NONE',  ( -110.8525252644344903, -292.7540674509536416, -254.6099447103820523 ) ) ;
#22680=CARTESIAN_POINT ( 'NONE',  ( 82.16961421606863780, -297.9242554544695736, -194.1646132934808406 ) ) ;
#22682=CARTESIAN_POINT ( 'NONE',  ( -98.25275556860052006, -275.1346827293161823, -225.9095922126304856 ) ) ;
#22683=CARTESIAN_POINT ( 'NONE',  ( 35.58909546793568524, -280.8337438970376070, -276.7754495574499742 ) ) ;
#22684=CARTESIAN_POINT ( 'NONE',  ( -69.89980877123716141, -281.4807601703192859, -337.9398652197405113 ) ) ;
#22685=CARTESIAN_POINT ( 'NONE',  ( -4.580679678801258703, -293.8286225840001293, -339.8800480576171026 ) ) ;
#22686=CARTESIAN_POINT ( 'NONE',  ( -111.3541991716151642, -270.8282264253883795, -267.5770889151806955 ) ) ;
#22687=CARTESIAN_POINT ( 'NONE',  ( 36.45115243676555394, -273.5052900686502539, -260.5667773727956842 ) ) ;
#22688=CARTESIAN_POINT ( 'NONE',  ( -71.91168270471584378, -298.9002826349354223, -205.4919094356256721 ) ) ;
#22690=CARTESIAN_POINT ( 'NONE',  ( -67.84030759116568277, -293.6868567188345764, -339.9585960872456099 ) ) ;
#22691=CARTESIAN_POINT ( 'NONE',  ( 31.14051418945081551, -295.3363995764118499, -297.4368706813414747 ) ) ;
#22693=CARTESIAN_POINT ( 'NONE',  ( -88.60772221111855629, -296.5964796720023742, -322.6280579143527234 ) ) ;
#22695=CARTESIAN_POINT ( 'NONE',  ( -107.7747926669414085, -282.2241158388961253, -297.2944512803562134 ) ) ;
#22696=CARTESIAN_POINT ( 'NONE',  ( -104.7622094669633697, -296.9275086513180213, -242.3704959729346058 ) ) ;
#22697=CARTESIAN_POINT ( 'NONE',  ( -93.91973698330325249, -285.2639561508167958, -218.0534269499433719 ) ) ;
#22698=CARTESIAN_POINT ( 'NONE',  ( -11.17728241618123519, -284.6341085752313234, -341.3020947738959876 ) ) ;
#22700=CARTESIAN_POINT ( 'NONE',  ( 22.07656087008093948, -286.5611476350845237, -221.4201887760816021 ) ) ;
#22701=CARTESIAN_POINT ( 'NONE',  ( -36.15206223956474929, -290.0669091157924413, -195.5244473746655842 ) ) ;
#22702=CARTESIAN_POINT ( 'NONE',  ( -113.6661288190491490, -277.7780515762037226, -280.1582730972108379 ) ) ;
#22703=CARTESIAN_POINT ( 'NONE',  ( 31.95455697924147387, -279.4809262143061233, -303.7686719486574134 ) ) ;
#22705=CARTESIAN_POINT ( 'NONE',  ( 32.68786815095917575, -286.6387749859839573, -292.5071935587822622 ) ) ;
#22706=CARTESIAN_POINT ( 'NONE',  ( -51.64120287927517694, -288.1512942791672458, -345.7070981672038101 ) ) ;
#22708=CARTESIAN_POINT ( 'NONE',  ( -95.68742849930090699, -279.3073181899726478, -319.7207665702244412 ) ) ;
#22709=CARTESIAN_POINT ( 'NONE',  ( -0.2906709608072832740, -292.5821596727428755, -335.9932554481637794 ) ) ;
#22710=CARTESIAN_POINT ( 'NONE',  ( 17.98332403503773236, -280.5401447333096598, -222.6845076996868045 ) ) ;
#22711=CARTESIAN_POINT ( 'NONE',  ( 36.37030796215024253, -294.0002845385174055, -292.8024803949475086 ) ) ;
#22712=CARTESIAN_POINT ( 'NONE',  ( -13.14133122367220352, -284.4439798700079791, -198.7813977996833898 ) ) ;
#22713=CARTESIAN_POINT ( 'NONE',  ( -110.1506655130680343, -280.7840555642916343, -252.3123750123670277 ) ) ;
#22714=CARTESIAN_POINT ( 'NONE',  ( -53.21200778094138428, -294.3192846342348616, -341.9083191063643312 ) ) ;
#22717=CARTESIAN_POINT ( 'NONE',  ( 23.43846087917011545, -282.9400340136804743, -227.0296186757534258 ) ) ;
#22718=CARTESIAN_POINT ( 'NONE',  ( -108.2331318604038017, -296.2934583097169252, -252.6352646284919956 ) ) ;
#22720=CARTESIAN_POINT ( 'NONE',  ( 21.27581636871891391, -273.6952119285918457, -317.1477375740089997 ) ) ;
#22721=CARTESIAN_POINT ( 'NONE',  ( 19.92237808443723424, -274.0523202826550460, -219.0483142096312008 ) ) ;
#22722=CARTESIAN_POINT ( 'NONE',  ( -70.21881600624524822, -291.4396067079047725, -205.1837042868152992 ) ) ;
#22723=CARTESIAN_POINT ( 'NONE',  ( -106.1687192835454852, -280.4223590243038871, -243.8827697135520225 ) ) ;
#22724=CARTESIAN_POINT ( 'NONE',  ( -40.83296186252206184, -275.6077761908522916, -196.5934976232818769 ) ) ;
#22725=CARTESIAN_POINT ( 'NONE',  ( -66.25364234098209693, -285.0244795096454595, -340.8772114131485296 ) ) ;
#22727=CARTESIAN_POINT ( 'NONE',  ( 35.96172176885659155, -280.3957013810674539, -274.0677123757845948 ) ) ;
#22728=CARTESIAN_POINT ( 'NONE',  ( -32.26029003107166915, -278.9883586160660229, -345.2401208762206579 ) ) ;
#22730=CARTESIAN_POINT ( 'NONE',  ( -13.06047496500069371, -274.1924623411498487, -197.2897685419343361 ) ) ;
#22731=CARTESIAN_POINT ( 'NONE',  ( -65.90161194582250914, -293.5957480110473057, -201.6040033838448267 ) ) ;
#22732=DIRECTION ( 'NONE',  ( -1.000000000000000000, -0.000000000000000000, -0.000000000000000000 ) ) ;
#22735=CARTESIAN_POINT ( 'NONE',  ( -19.59989027179562271, -292.9660803456000622, -344.0733412432311411 ) ) ;
#22736=CARTESIAN_POINT ( 'NONE',  ( 17.33577515472369512, -274.3672531237997987, -221.8262426903179119 ) ) ;
#22738=CARTESIAN_POINT ( 'NONE',  ( 10.66741075741771816, -294.2216001917107064, -210.9818282037762458 ) ) ;
#22739=CARTESIAN_POINT ( 'NONE',  ( 21.31550574532285580, -278.6948066931273615, -317.0979686699210447 ) ) ;
#22740=CARTESIAN_POINT ( 'NONE',  ( -72.00637819585742250, -292.8091966474985952, -202.0357678544988573 ) ) ;
#22741=CARTESIAN_POINT ( 'NONE',  ( 4.664257116669503489, -290.4842402642510706, -332.3552547765065128 ) ) ;
#22742=CARTESIAN_POINT ( 'NONE',  ( -15.87882209927194488, -274.7738702344745434, -342.1048748589603861 ) ) ;
#22743=CARTESIAN_POINT ( 'NONE',  ( 3.952851430080756678, -278.4113567900880071, -332.2971673211025632 ) ) ;
#22744=CARTESIAN_POINT ( 'NONE',  ( 36.85786856815133206, -291.7093286840240012, -276.3392616079703998 ) ) ;
#22745=CARTESIAN_POINT ( 'NONE',  ( -69.46064954653174084, -281.4944336589909994, -201.7271460564375047 ) ) ;
#22747=CARTESIAN_POINT ( 'NONE',  ( -13.52647936258182426, -282.4011125619427958, -339.4431566570673908 ) ) ;
#22748=CARTESIAN_POINT ( 'NONE',  ( -33.94278438221868299, -281.1736391956857801, -193.7455850789679914 ) ) ;
#22749=CARTESIAN_POINT ( 'NONE',  ( 23.92823234629980433, -280.9622221717011143, -316.3394182371355328 ) ) ;
#22750=CARTESIAN_POINT ( 'NONE',  ( 14.73239419996653332, -277.2815191724564556, -326.8347959583882130 ) ) ;
#22752=CARTESIAN_POINT ( 'NONE',  ( 26.34117372993448924, -276.5144197671795609, -228.3230479796506529 ) ) ;
#22754=CARTESIAN_POINT ( 'NONE',  ( -53.28691492658256834, -291.7662352645559167, -340.3683826091709079 ) ) ;
#22756=B_SPLINE_CURVE_WITH_KNOTS ( 'NONE', 3,
 ( #32652, #34051, #26476, #10846, #69559, #4688, #39710, #77604, #3767, #40181 ),
 .UNSPECIFIED., .F., .F.,
 ( 4, 2, 2, 2, 4 ),
 ( 0.000000000000000000, 0.04477231361816515209, 0.08954462723633030419, 0.1343169408544954702, 0.1790892544726606084 ),
 .UNSPECIFIED. ) ;
#22758=CARTESIAN_POINT ( 'NONE',  ( -68.91200057829905745, -299.6372711141936520, -202.3153437795381535 ) ) ;
#22760=CARTESIAN_POINT ( 'NONE',  ( -30.79299449257197807, -293.2165522940872506, -197.3450887278570463 ) ) ;
#22761=CARTESIAN_POINT ( 'NONE',  ( -97.43176018785064230, -275.9650703533350793, -314.6660869604590403 ) ) ;
#22762=CARTESIAN_POINT ( 'NONE',  ( -97.55915349704285688, -292.9391401709866045, -223.9953431056200941 ) ) ;
#22763=CARTESIAN_POINT ( 'NONE',  ( -28.08522986115089637, -291.5211917964301733, -197.7967795870209784 ) ) ;
#22764=EDGE_CURVE ( 'NONE', #16725, #72158, #12429, .T. ) ;
#22765=CARTESIAN_POINT ( 'NONE',  ( -1.834701946944296225, -288.1021422454562071, -338.6163740701982192 ) ) ;
#22767=CARTESIAN_POINT ( 'NONE',  ( 34.90151646025780963, -291.8089060723391412, -245.3106039014988937 ) ) ;
#22768=CARTESIAN_POINT ( 'NONE',  ( -64.36709589736504711, -281.8107076448854400, -339.0347548387805432 ) ) ;
#22769=CARTESIAN_POINT ( 'NONE',  ( -93.32793867447479386, -291.7283439639663811, -319.1863069001528288 ) ) ;
#22770=CARTESIAN_POINT ( 'NONE',  ( -109.8720068664262755, -283.2033640286816762, -257.2494340120659331 ) ) ;
#22771=CARTESIAN_POINT ( 'NONE',  ( -64.22024288570915473, -284.7255395279689196, -338.7627803713127719 ) ) ;
#22773=CARTESIAN_POINT ( 'NONE',  ( -40.31759989762937835, -290.0299206082618753, -347.0811623483997437 ) ) ;
#22774=CARTESIAN_POINT ( 'NONE',  ( -16.91050925244443448, -280.8155941523984325, -200.2144510560181345 ) ) ;
#22775=CARTESIAN_POINT ( 'NONE',  ( -13.97290882141705914, -291.1435456870715370, -197.3540172353421269 ) ) ;
#22776=CARTESIAN_POINT ( 'NONE',  ( -12.76505267549691958, -287.1665277195018575, -197.5590079843245519 ) ) ;
#22777=CARTESIAN_POINT ( 'NONE',  ( 34.79435364268214670, -287.7059417146654141, -243.6044991845759284 ) ) ;
#22778=CARTESIAN_POINT ( 'NONE',  ( -97.35715053496559790, -285.2980992667718851, -228.7800786883462933 ) ) ;
#22781=CARTESIAN_POINT ( 'NONE',  ( 27.06853868113006456, -295.9439221579730770, -310.3549262581429389 ) ) ;
#22782=CARTESIAN_POINT ( 'NONE',  ( -33.47660968079976840, -293.6893154319278096, -346.7833109541220438 ) ) ;
#22783=CARTESIAN_POINT ( 'NONE',  ( -79.17950020349032059, -278.5307175752861895, -210.2528246079047847 ) ) ;
#22784=CARTESIAN_POINT ( 'NONE',  ( -89.53302443627046614, -296.6883992669565941, -213.8144110142056036 ) ) ;
#22785=CARTESIAN_POINT ( 'NONE',  ( -0.8971089609653338792, -291.0252516736392181, -206.2957458962374631 ) ) ;
#22786=CARTESIAN_POINT ( 'NONE',  ( -111.0574343037965406, -294.8854469085159167, -263.1793407518790673 ) ) ;
#22787=CARTESIAN_POINT ( 'NONE',  ( 33.83486101183537897, -294.9924159393723926, -288.2783624762129193 ) ) ;
#22788=CARTESIAN_POINT ( 'NONE',  ( 34.24870465095800398, -294.4237640906870297, -254.5221191405164802 ) ) ;
#22790=CARTESIAN_POINT ( 'NONE',  ( 0.8162758624145598496, -292.5442274639501079, -335.1221965322361029 ) ) ;
#22791=CARTESIAN_POINT ( 'NONE',  ( -101.4668613245127347, -298.0298803328688564, -309.3560345559305915 ) ) ;
#22792=CARTESIAN_POINT ( 'NONE',  ( -108.3395303076698326, -291.7303467748802746, -252.3457680708250450 ) ) ;
#22794=CARTESIAN_POINT ( 'NONE',  ( -69.72963153454597318, -295.8241083238206102, -335.8065867797317878 ) ) ;
#22795=ADVANCED_FACE ( 'NONE', ( #3461 ), #59853, .F. ) ;
#22796=CARTESIAN_POINT ( 'NONE',  ( -110.8737549414448438, -280.3214923827876532, -286.8366672158840629 ) ) ;
#22797=CARTESIAN_POINT ( 'NONE',  ( -110.8587005888958146, -277.5042360618326711, -249.1821445290698591 ) ) ;
#22799=CARTESIAN_POINT ( 'NONE',  ( -102.6281135752596612, -272.4330257089519023, -229.7286555217281148 ) ) ;
#22800=CARTESIAN_POINT ( 'NONE',  ( -0.5613685635308771626, -280.6391429359832728, -335.0799051208878154 ) ) ;
#22801=CARTESIAN_POINT ( 'NONE',  ( -113.5770022875950360, -276.9726275541875680, -268.7308133519520652 ) ) ;
#22802=CARTESIAN_POINT ( 'NONE',  ( -25.65490631274033007, -278.2005651184741737, -196.1085269536625901 ) ) ;
#22803=CARTESIAN_POINT ( 'NONE',  ( -68.23968605179433666, -296.3224740033879243, -203.6648462538233275 ) ) ;
#22804=CARTESIAN_POINT ( 'NONE',  ( -11.88347930468330205, -276.3835672010429789, -199.7597039274096744 ) ) ;
#22806=CARTESIAN_POINT ( 'NONE',  ( -111.0262047432414505, -288.7746597923503487, -254.5205847825237697 ) ) ;
#22807=CARTESIAN_POINT ( 'NONE',  ( -36.08684223591867379, -289.0368599404415590, -347.3640025296235194 ) ) ;
#22808=CARTESIAN_POINT ( 'NONE',  ( 33.98207351173908108, -277.2444477820234283, -246.4706957618994636 ) ) ;
#22809=CARTESIAN_POINT ( 'NONE',  ( -44.72524722593194468, -295.9584584440430035, -195.8412787701375635 ) ) ;
#22810=CARTESIAN_POINT ( 'NONE',  ( -32.30676869908135274, -285.3112654799778056, -193.6745922750766340 ) ) ;
#22811=DIRECTION ( 'NONE',  ( 0.000000000000000000, -1.000000000000000000, 0.000000000000000000 ) ) ;
#22812=CARTESIAN_POINT ( 'NONE',  ( 35.63726443635285079, -279.7746893963228558, -287.7093475087763750 ) ) ;
#22815=CARTESIAN_POINT ( 'NONE',  ( 29.10448190937588109, -291.9267881195015661, -239.0636326948262820 ) ) ;
#22816=CARTESIAN_POINT ( 'NONE',  ( -84.41310688868244938, -283.5362906318811156, -212.8909640408337793 ) ) ;
#22819=CARTESIAN_POINT ( 'NONE',  ( 35.59865740017828273, -291.3272050173316075, -252.8503742251963047 ) ) ;
#22820=CARTESIAN_POINT ( 'NONE',  ( -110.9648532524177966, -280.0765960735530484, -276.1618340421539415 ) ) ;
#22821=CARTESIAN_POINT ( 'NONE',  ( -71.54759087307321863, -284.6990428877417116, -338.9028261502468808 ) ) ;
#22822=CARTESIAN_POINT ( 'NONE',  ( -21.62990425952631668, -272.3319021090456431, -196.4527039436227938 ) ) ;
#22823=CARTESIAN_POINT ( 'NONE',  ( -106.5323114736921326, -284.8631950325906814, -246.9292609112477805 ) ) ;
#22824=( BOUNDED_CURVE ( )  B_SPLINE_CURVE ( 3, ( #59992, #22581, #30163, #66616 ),
 .UNSPECIFIED., .F., .F. ) 
 B_SPLINE_CURVE_WITH_KNOTS ( ( 4, 4 ),
 ( 1.570796326794433151, 4.712388980385153303 ),
 .UNSPECIFIED. ) 
 CURVE ( )  GEOMETRIC_REPRESENTATION_ITEM ( )  RATIONAL_B_SPLINE_CURVE ( ( 1.000000000000000000, 0.3333333333330242843, 0.3333333333330242843, 1.000000000000000000 ) ) 
 REPRESENTATION_ITEM ( '' )  );
#22825=CARTESIAN_POINT ( 'NONE',  ( 28.37943907704037727, -276.5316721041541541, -237.2536146483415678 ) ) ;
#22826=CARTESIAN_POINT ( 'NONE',  ( -7.432304353985270673, -277.4524491857194448, -337.1295968617869789 ) ) ;
#22827=CARTESIAN_POINT ( 'NONE',  ( -102.3207591046432583, -287.0533518841056662, -232.8048436453463239 ) ) ;
#22830=CARTESIAN_POINT ( 'NONE',  ( -113.2042502678440741, -296.2167936307116065, -283.8485727529573523 ) ) ;
#22832=CARTESIAN_POINT ( 'NONE',  ( 19.00151691237411100, -288.8493686725484508, -221.3990030523627013 ) ) ;
#22834=CARTESIAN_POINT ( 'NONE',  ( -119.3990491898856732, -294.0523547857346784, -270.3284710469131937 ) ) ;
#22835=CARTESIAN_POINT ( 'NONE',  ( -98.32217382835952435, -278.0952094886043824, -223.8330176317634255 ) ) ;
#22836=CARTESIAN_POINT ( 'NONE',  ( -16.82225183866680496, -290.7127568243128053, -196.9758833949151438 ) ) ;
#22838=CARTESIAN_POINT ( 'NONE',  ( 34.69248652820068912, -289.2761949266253509, -285.9697713353139648 ) ) ;
#22839=CARTESIAN_POINT ( 'NONE',  ( -106.4686551089934170, -280.6623396288676986, -243.7705632818004062 ) ) ;
#22840=CARTESIAN_POINT ( 'NONE',  ( 7.602705703670109116, -289.8777964016595092, -332.2212524178387412 ) ) ;
#22841=CARTESIAN_POINT ( 'NONE',  ( 11.22261843696981209, -284.3800312508116122, -327.5828045920850400 ) ) ;
#22842=CARTESIAN_POINT ( 'NONE',  ( -89.21054873758203030, -277.9251035745185163, -327.2700149004718924 ) ) ;
#22843=CARTESIAN_POINT ( 'NONE',  ( -67.46039558916896794, -295.6752633816268485, -202.0484428998865667 ) ) ;
#22844=CARTESIAN_POINT ( 'NONE',  ( -69.96044476446304827, -279.4676661538749727, -200.5970513612901414 ) ) ;
#22845=CARTESIAN_POINT ( 'NONE',  ( -67.58200756528542286, -275.5115775192335263, -202.5505148680412049 ) ) ;
#22847=CARTESIAN_POINT ( 'NONE',  ( 21.27581636871892101, -289.4090924074130839, -223.5744983911110353 ) ) ;
#22848=EDGE_CURVE ( 'NONE', #21957, #32677, #6490, .T. ) ;
#22849=CARTESIAN_POINT ( 'NONE',  ( -98.73490887853469644, -271.3952536205675301, -225.4983732049233254 ) ) ;
#22851=CARTESIAN_POINT ( 'NONE',  ( -57.12385550252515287, -279.2975952226574918, -200.0286591159144791 ) ) ;
#22852=CARTESIAN_POINT ( 'NONE',  ( 28.15503812785641102, -276.2348025467925368, -230.5333556394868140 ) ) ;
#22853=CARTESIAN_POINT ( 'NONE',  ( -31.66568236574773110, -282.0409348993216554, -346.9289209039087041 ) ) ;
#22854=CARTESIAN_POINT ( 'NONE',  ( -56.30387553490361086, -291.0598309202619589, -341.9574636689927729 ) ) ;
#22855=CARTESIAN_POINT ( 'NONE',  ( -98.54800878943147779, -298.6840714951786140, -224.7707226745167475 ) ) ;
#22856=CARTESIAN_POINT ( 'NONE',  ( -3.643216289488539594, -299.6703060159638881, -193.7514583082898980 ) ) ;
#22857=CARTESIAN_POINT ( 'NONE',  ( 36.12906626429139578, -295.7352411283621905, -284.5764236440898003 ) ) ;
#22858=CARTESIAN_POINT ( 'NONE',  ( 34.88970170094819423, -279.2993518203380745, -250.7505102836038873 ) ) ;
#22859=CARTESIAN_POINT ( 'NONE',  ( -8.308312740321206036, -272.4541422371714248, -201.5389169675738117 ) ) ;
#22860=CARTESIAN_POINT ( 'NONE',  ( 23.21315494456706574, -288.5288294261599162, -224.0844620599828261 ) ) ;
#22862=CARTESIAN_POINT ( 'NONE',  ( -80.60094962465606727, -288.5743577796425825, -329.6092881494023459 ) ) ;
#22863=CARTESIAN_POINT ( 'NONE',  ( 204.7385621006099257, 294.9048254156659823, -54.00000000002585665 ) ) ;
#22865=CARTESIAN_POINT ( 'NONE',  ( -62.58624418680784629, -287.9489336413535057, -342.5372485129394704 ) ) ;
#22866=CARTESIAN_POINT ( 'NONE',  ( 21.97639084872056614, -287.8140071819120180, -312.9457580501953089 ) ) ;
#22867=ORIENTED_EDGE ( 'NONE', *, *, #45976, .T. ) ;
#22868=CARTESIAN_POINT ( 'NONE',  ( -37.99366749977676960, -287.1238288974059856, -193.6729999342475423 ) ) ;
#22869=CARTESIAN_POINT ( 'NONE',  ( -6.263773649677868427, -276.9655234373737471, -336.4524965866945081 ) ) ;
#22870=CARTESIAN_POINT ( 'NONE',  ( -6.000628894711874217, -291.3748327941144112, -200.3523874316296371 ) ) ;
#22871=CARTESIAN_POINT ( 'NONE',  ( -1.674044572686927523, -283.2434110234169680, -338.4869657503185181 ) ) ;
#22872=CARTESIAN_POINT ( 'NONE',  ( 12.52433140809071865, -282.2526717859820451, -212.6022515651207812 ) ) ;
#22873=CARTESIAN_POINT ( 'NONE',  ( -67.86906395222227673, -283.7753189327724499, -341.0281141655796091 ) ) ;
#22874=CARTESIAN_POINT ( 'NONE',  ( -41.05650413763851247, -280.3373952814051222, -197.4345266869805755 ) ) ;
#22875=CARTESIAN_POINT ( 'NONE',  ( -114.2704648735229114, -276.0523547857348490, -270.3284710469133074 ) ) ;
#22876=CARTESIAN_POINT ( 'NONE',  ( -107.5233622349960143, -262.7998339567401445, -317.7199647377577776 ) ) ;
#22878=CARTESIAN_POINT ( 'NONE',  ( -96.71237328335487859, -279.9270754022212486, -315.9149498662736733 ) ) ;
#22879=CARTESIAN_POINT ( 'NONE',  ( -84.92918389587137540, -218.7266517812545601, -351.7339122337344861 ) ) ;
#22880=CARTESIAN_POINT ( 'NONE',  ( 83.26066877736924710, 82.48078560638359136, -299.1889401045851287 ) ) ;
#22881=CARTESIAN_POINT ( 'NONE',  ( -37.81486326515116758, -297.3946560319042192, -197.2607158959976346 ) ) ;
#22882=CARTESIAN_POINT ( 'NONE',  ( 28.05031060861441361, -293.5915381554420946, -311.0002138651627206 ) ) ;
#22883=CARTESIAN_POINT ( 'NONE',  ( -110.5520848501708855, -271.4739283423095344, -283.6991303856082709 ) ) ;
#22884=CARTESIAN_POINT ( 'NONE',  ( -108.7005367908344198, -271.5903782609459540, -242.6252554518754607 ) ) ;
#22885=CARTESIAN_POINT ( 'NONE',  ( -109.1333380604779109, -288.7288743595184997, -287.4608589319041698 ) ) ;
#22886=CARTESIAN_POINT ( 'NONE',  ( -106.0971639671342928, -298.0438304111626735, -298.3531109505069026 ) ) ;
#22887=CARTESIAN_POINT ( 'NONE',  ( -8.006353524199305127, -289.9749296745324614, -337.8001041016131012 ) ) ;
#22889=CARTESIAN_POINT ( 'NONE',  ( 8.774395754089230337, -295.3782415246955111, -331.7298878324195357 ) ) ;
#22890=CARTESIAN_POINT ( 'NONE',  ( 0.1949017428794037610, -287.0585737428667699, -207.6204676616511904 ) ) ;
#22891=CARTESIAN_POINT ( 'NONE',  ( -48.89487286685766065, -296.7031806015959887, -194.5810305377431746 ) ) ;
#22892=CARTESIAN_POINT ( 'NONE',  ( 1.609407422514420372, -293.3614706655782811, -204.0661102242755192 ) ) ;
#22893=CARTESIAN_POINT ( 'NONE',  ( 29.41913012166305563, -293.5472216982245754, -232.1182304418038029 ) ) ;
#22894=CARTESIAN_POINT ( 'NONE',  ( -36.20825930646101654, -292.2333990132634085, -197.3574412278100567 ) ) ;
#22896=CARTESIAN_POINT ( 'NONE',  ( -111.0442044302446618, -274.6845124885824134, -253.7101401615071836 ) ) ;
#22897=CARTESIAN_POINT ( 'NONE',  ( 38.10372819436256009, -274.1793635155243578, -257.0197307579413746 ) ) ;
#22899=CARTESIAN_POINT ( 'NONE',  ( -5.316111143675319006, -276.1495667217936898, -340.3174511746917119 ) ) ;
#22900=CARTESIAN_POINT ( 'NONE',  ( -107.9560938384698261, -271.2350164550532554, -248.7375006393052672 ) ) ;
#22901=CARTESIAN_POINT ( 'NONE',  ( -13.40922665110629453, -274.8777730879430123, -340.6867792316156738 ) ) ;
#22902=CARTESIAN_POINT ( 'NONE',  ( 95.29650580809318683, -300.9540312850523378, -196.9362300929560945 ) ) ;
#22903=CARTESIAN_POINT ( 'NONE',  ( -29.97808937807558038, -275.0888931880960513, -197.4969588592658738 ) ) ;
#22904=CARTESIAN_POINT ( 'NONE',  ( -9.495033719286549712, -299.9954019213857919, -194.1536752346991648 ) ) ;
#22906=CARTESIAN_POINT ( 'NONE',  ( -80.29176131480143397, -271.4941183381000087, -208.3810282358067241 ) ) ;
#22907=CARTESIAN_POINT ( 'NONE',  ( -58.42972677395699321, -295.9835123121719107, -340.3553163143595839 ) ) ;
#22908=CARTESIAN_POINT ( 'NONE',  ( -12.82894162297253082, -293.3020599748949735, -339.8013953134497456 ) ) ;
#22910=CARTESIAN_POINT ( 'NONE',  ( 18.86254208852871272, -276.7616678237225756, -322.9026259556976584 ) ) ;
#22912=CARTESIAN_POINT ( 'NONE',  ( -48.87752903021296191, -274.0679296571243526, -198.2271817964278853 ) ) ;
#22913=CARTESIAN_POINT ( 'NONE',  ( -112.6545574498353517, -283.0638493678085297, -284.1160664332224997 ) ) ;
#22914=CARTESIAN_POINT ( 'NONE',  ( -66.19653985408517372, -297.4290927373858722, -339.7826635079074435 ) ) ;
#22916=CARTESIAN_POINT ( 'NONE',  ( -67.60517963137860420, -284.8417675753788103, -203.7523833015337118 ) ) ;
#22917=CARTESIAN_POINT ( 'NONE',  ( -96.09085878621074528, -276.1673820875641354, -315.3778967769584938 ) ) ;
#22918=CARTESIAN_POINT ( 'NONE',  ( -109.8698891021753639, -276.9629605387547713, -282.8870801509284547 ) ) ;
#22919=CARTESIAN_POINT ( 'NONE',  ( -12.09036619058301376, -284.7238632199299673, -341.0363372823140367 ) ) ;
#22920=CARTESIAN_POINT ( 'NONE',  ( 33.89085614128760682, -276.5250112258291892, -252.6678019186929305 ) ) ;
#22922=CARTESIAN_POINT ( 'NONE',  ( 29.82814540138188519, -274.4232409526422884, -306.4537523632698708 ) ) ;
#22923=CARTESIAN_POINT ( 'NONE',  ( -12.14840405729502137, -282.3792223695888310, -199.4875086002994919 ) ) ;
#22925=CARTESIAN_POINT ( 'NONE',  ( 17.29305766490441698, -288.7442011317996275, -218.0903091792585258 ) ) ;
#22927=CARTESIAN_POINT ( 'NONE',  ( -102.1350131748652927, -288.0462287910465875, -308.2362795624047749 ) ) ;
#22929=CARTESIAN_POINT ( 'NONE',  ( -35.78972779189328435, -296.8669275165477757, -196.9643687994915524 ) ) ;
#22930=CARTESIAN_POINT ( 'NONE',  ( -111.3561666106230632, -288.6093401080416356, -276.7123986008949146 ) ) ;
#22931=CARTESIAN_POINT ( 'NONE',  ( 61.48257290429442889, 47.14312216093964025, -312.8229988924202871 ) ) ;
#22933=CARTESIAN_POINT ( 'NONE',  ( 22.46070306245089299, -285.3918514258581922, -222.9442895481464859 ) ) ;
#22934=CARTESIAN_POINT ( 'NONE',  ( -48.42897952224370073, -284.7957664921333389, -343.3235237083409856 ) ) ;
#22935=CARTESIAN_POINT ( 'NONE',  ( -80.34600888977716693, -283.7185653825162035, -207.6509628155010034 ) ) ;
#22936=CARTESIAN_POINT ( 'NONE',  ( 17.48982983209532449, -282.2808244831265370, -221.2807936141313121 ) ) ;
#22937=CARTESIAN_POINT ( 'NONE',  ( 20.31452793060773487, -282.9883822624314007, -315.3984479830546093 ) ) ;
#22938=CARTESIAN_POINT ( 'NONE',  ( -34.69870929487166222, -290.9989806303004798, -345.6699581337700806 ) ) ;
#22939=CARTESIAN_POINT ( 'NONE',  ( -94.13253428802087797, -273.5926075519712413, -218.3748818926861475 ) ) ;
#22940=CARTESIAN_POINT ( 'NONE',  ( 31.54190348104442165, -286.0362430933452060, -301.4153181661799863 ) ) ;
#22941=CARTESIAN_POINT ( 'NONE',  ( 4.863160820755996205, -274.6050010984182563, -205.8948307274026490 ) ) ;
#22942=CARTESIAN_POINT ( 'NONE',  ( 36.46817474507574275, -295.6800233298317835, -281.8313114947656572 ) ) ;
#22944=CARTESIAN_POINT ( 'NONE',  ( 31.03373250439201669, -301.4082689599840705, -195.3320873922940848 ) ) ;
#22945=CARTESIAN_POINT ( 'NONE',  ( -66.77233571673012591, -282.1308321146674416, -337.7177936702101420 ) ) ;
#22946=CARTESIAN_POINT ( 'NONE',  ( -112.5509510421484407, -276.5367145921179599, -271.5532795534923025 ) ) ;
#22947=CARTESIAN_POINT ( 'NONE',  ( -91.66179662871803657, -271.7748953214217522, -216.7697486382825502 ) ) ;
#22948=CARTESIAN_POINT ( 'NONE',  ( 31.21678539507831829, -274.5629146278374719, -244.9913184014182832 ) ) ;
#22949=CARTESIAN_POINT ( 'NONE',  ( -14.65113616183396950, -293.8717674158717159, -200.2480232123132566 ) ) ;
#22950=CARTESIAN_POINT ( 'NONE',  ( 35.07247113035655417, -294.6415507602708885, -281.6273338381378721 ) ) ;
#22951=CARTESIAN_POINT ( 'NONE',  ( -111.3228750145086394, -286.3406870128762876, -268.1794274846537860 ) ) ;
#22952=CARTESIAN_POINT ( 'NONE',  ( 8.482944460584493029, -294.0908240747454556, -209.1501151698160186 ) ) ;
#22953=CARTESIAN_POINT ( 'NONE',  ( 39.16223351306230427, -294.8305394199445004, -267.4386253259762043 ) ) ;
#22954=CARTESIAN_POINT ( 'NONE',  ( -109.0452700252175049, -296.5670311119403095, -256.5979082342217907 ) ) ;
#22955=CARTESIAN_POINT ( 'NONE',  ( -111.1425255844403210, -292.3807953661203669, -283.7192171284036704 ) ) ;
#22956=CARTESIAN_POINT ( 'NONE',  ( -111.8744294936991679, -284.4762362498173047, -289.7491621985259940 ) ) ;
#22957=CARTESIAN_POINT ( 'NONE',  ( -72.58675008682091345, -295.6695041169023739, -203.4670124633767045 ) ) ;
#22958=CARTESIAN_POINT ( 'NONE',  ( -114.2084971262152067, -284.3185065081116818, -275.7156657377469173 ) ) ;
#22959=CARTESIAN_POINT ( 'NONE',  ( -24.01165265740753085, -278.8610975586097993, -343.8586529574663473 ) ) ;
#22960=CARTESIAN_POINT ( 'NONE',  ( -91.80561436760662275, -284.0486309817471806, -221.0847036836681241 ) ) ;
#22961=CARTESIAN_POINT ( 'NONE',  ( 36.99639573262543735, -285.4243330106365306, -260.4188771728639722 ) ) ;
#22962=CARTESIAN_POINT ( 'NONE',  ( -53.47399151803750783, -277.9870680884278045, -196.2800364275581728 ) ) ;
#22963=CARTESIAN_POINT ( 'NONE',  ( 202.9738562182569694, 296.4636489450776367, -53.99999999999997868 ) ) ;
#22965=CARTESIAN_POINT ( 'NONE',  ( -81.51080159783965939, -284.9400560793508248, -212.1625018751630591 ) ) ;
#22967=CARTESIAN_POINT ( 'NONE',  ( 39.13381660647873872, -282.8233149462358256, -275.6182787201078099 ) ) ;
#22968=CARTESIAN_POINT ( 'NONE',  ( -5.734359013657527093, -287.7053336863788786, -340.3167911008455917 ) ) ;
#22969=CARTESIAN_POINT ( 'NONE',  ( -86.56274151179913190, -279.3225764183724777, -328.5999738795804888 ) ) ;
#22970=CARTESIAN_POINT ( 'NONE',  ( 7.962606359018053581, -277.7629737672214674, -332.0774945443131401 ) ) ;
#22971=CARTESIAN_POINT ( 'NONE',  ( -54.49072983551907612, -279.6590751916525051, -199.3518160029029787 ) ) ;
#22972=CARTESIAN_POINT ( 'NONE',  ( -18.88886148336236559, -276.2706384674692686, -197.9795143481037485 ) ) ;
#22973=CARTESIAN_POINT ( 'NONE',  ( 35.48641470901812056, -293.8690876775477250, -295.5258246053791140 ) ) ;
#22974=CARTESIAN_POINT ( 'NONE',  ( 33.11721102769511305, -285.8794511299716419, -295.5716368973623958 ) ) ;
#22976=CARTESIAN_POINT ( 'NONE',  ( -53.24248247744834828, -293.4518036238951026, -195.7846667730574097 ) ) ;
#22977=CARTESIAN_POINT ( 'NONE',  ( -35.65723826049037370, -293.9508856762885216, -343.6634254068538894 ) ) ;
#22978=CARTESIAN_POINT ( 'NONE',  ( 1.577513483448755194, -294.1832471369779114, -332.2059690744101772 ) ) ;
#22979=CARTESIAN_POINT ( 'NONE',  ( -74.54104606260183630, -292.6488187284438141, -203.2962152976063521 ) ) ;
#22980=CARTESIAN_POINT ( 'NONE',  ( 13.39989437834137753, -281.4362347407014795, -217.6675544099526292 ) ) ;
#22981=CARTESIAN_POINT ( 'NONE',  ( -113.9453354313073845, -271.6827742692142920, -264.6318282315379520 ) ) ;
#22982=CARTESIAN_POINT ( 'NONE',  ( 31.59971973709275161, -288.6432405057769301, -304.5457832979413411 ) ) ;
#22983=CARTESIAN_POINT ( 'NONE',  ( 16.92475570159112763, -280.4292092753884731, -323.3081412820886271 ) ) ;
#22984=CARTESIAN_POINT ( 'NONE',  ( -20.49689700323688513, -289.1749494576038728, -345.5289982074760928 ) ) ;
#22985=CARTESIAN_POINT ( 'NONE',  ( -25.14246470401097255, -286.5451444338183364, -198.3149018609613847 ) ) ;
#22986=CARTESIAN_POINT ( 'NONE',  ( 160.7988830096749382, 220.5294184115326459, -205.1624142896263550 ) ) ;
#22987=CARTESIAN_POINT ( 'NONE',  ( -78.98035441448926974, -207.4150709411190689, -355.2989178682290685 ) ) ;
#22988=CARTESIAN_POINT ( 'NONE',  ( 188.5977483363980127, 268.2578132117691894, -137.4814016061846189 ) ) ;
#22989=CARTESIAN_POINT ( 'NONE',  ( -95.73446723578864237, -278.3673783251171017, -226.2621407561551052 ) ) ;
#22990=CARTESIAN_POINT ( 'NONE',  ( -109.3494968692206868, -277.2909654271063005, -284.1789922881871462 ) ) ;
#22991=CARTESIAN_POINT ( 'NONE',  ( -96.91700721076711034, -272.8737681429720396, -221.5909131080033774 ) ) ;
#22992=CARTESIAN_POINT ( 'NONE',  ( 154.8888658863856165, 204.4229923944245684, -215.0313167292097205 ) ) ;
#22993=CARTESIAN_POINT ( 'NONE',  ( -59.11672987363058240, -278.3504499402774854, -197.1186823927174601 ) ) ;
#22994=CARTESIAN_POINT ( 'NONE',  ( 27.25644497146580392, -295.8436636034106755, -310.4731855529720406 ) ) ;
#22995=CARTESIAN_POINT ( 'NONE',  ( -72.66219300452470975, -292.0637266457310375, -206.3476288016925082 ) ) ;
#22996=CARTESIAN_POINT ( 'NONE',  ( -114.1068513207666797, -273.5291142825242332, -267.5143728961976990 ) ) ;
#22997=CARTESIAN_POINT ( 'NONE',  ( -76.14322411918233513, -288.2674159912355663, -332.7765424677062356 ) ) ;
#22998=CARTESIAN_POINT ( 'NONE',  ( -67.50331407874537604, -274.3181487566125156, -199.6250604822606078 ) ) ;
#22999=CARTESIAN_POINT ( 'NONE',  ( -102.5332902185967043, -297.1660282703861071, -237.3995630500442928 ) ) ;
#23001=CARTESIAN_POINT ( 'NONE',  ( -68.10898923914206193, -281.5714837469734562, -201.3347671768908640 ) ) ;
#23003=CARTESIAN_POINT ( 'NONE',  ( -109.4385882997463000, -279.8062272867600768, -257.0846429150424797 ) ) ;
#23004=CARTESIAN_POINT ( 'NONE',  ( -101.2326514894390357, -279.7642788576508792, -311.5900488088277598 ) ) ;
#23005=CARTESIAN_POINT ( 'NONE',  ( -6.218724311040165986, -272.9485804728112157, -203.5624044412007549 ) ) ;
#23008=CARTESIAN_POINT ( 'NONE',  ( -83.43938179525416388, -279.5666383645781821, -213.6917700477247024 ) ) ;
#23009=CARTESIAN_POINT ( 'NONE',  ( 31.71466012861212747, -276.7898872167788227, -304.1777121561370336 ) ) ;
#23010=CARTESIAN_POINT ( 'NONE',  ( 35.68162627385076746, -277.3320258031395156, -253.1999424596317283 ) ) ;
#23011=CARTESIAN_POINT ( 'NONE',  ( -113.1837301557192745, -277.0043172686608273, -280.0863615219236635 ) ) ;
#23014=CARTESIAN_POINT ( 'NONE',  ( 30.91350203915564521, -283.9512322764812211, -302.4158513194743705 ) ) ;
#23015=CARTESIAN_POINT ( 'NONE',  ( -101.2597868920018698, -290.2362179963678841, -234.6610229866321049 ) ) ;
#23017=CARTESIAN_POINT ( 'NONE',  ( -43.64962250782689779, -285.3231538857705800, -193.6690169835193558 ) ) ;
#23018=CARTESIAN_POINT ( 'NONE',  ( -74.32227712914057349, -281.7904756997564846, -334.5320164725492305 ) ) ;
#23019=CARTESIAN_POINT ( 'NONE',  ( -5.796700387507616625, -281.2038489659973379, -336.8602238486927831 ) ) ;
#23020=CARTESIAN_POINT ( 'NONE',  ( -6.617133361948789094, -281.6698648055175340, -203.6905802588781000 ) ) ;
#23021=CARTESIAN_POINT ( 'NONE',  ( 202.9737692353694740, 295.9636489105243413, -68.65455606434399272 ) ) ;
#23023=CARTESIAN_POINT ( 'NONE',  ( 13.13543902327948487, -280.7607650365613949, -327.5145976760659323 ) ) ;
#23024=CARTESIAN_POINT ( 'NONE',  ( 32.59592577037092553, -295.9046202721189616, -297.4485528984286020 ) ) ;
#23026=CARTESIAN_POINT ( 'NONE',  ( -59.98256321325585816, -287.7597293091604342, -198.6310622545221634 ) ) ;
#23027=CARTESIAN_POINT ( 'NONE',  ( 115.2448031289451222, -299.5541904835127980, -191.8695490883551713 ) ) ;
#23028=CARTESIAN_POINT ( 'NONE',  ( -95.48672851981423548, -293.1336711991844481, -222.0868933449800693 ) ) ;
#23030=CARTESIAN_POINT ( 'NONE',  ( -35.08222007661247943, -275.0236121215559706, -345.3270796028173777 ) ) ;
#23031=CARTESIAN_POINT ( 'NONE',  ( -71.84314555784575873, -288.6937545219195727, -339.0183032178874214 ) ) ;
#23032=CARTESIAN_POINT ( 'NONE',  ( 17.34455401813339748, -291.2489898442638037, -220.7295676744528521 ) ) ;
#23033=CARTESIAN_POINT ( 'NONE',  ( -71.90079450396511618, -276.2038635667711901, -335.2360302347020138 ) ) ;
#23034=CARTESIAN_POINT ( 'NONE',  ( -92.75133650044125488, -295.3864797292696949, -220.9583075494125239 ) ) ;
#23036=CARTESIAN_POINT ( 'NONE',  ( -71.38642831329084970, -290.8267312493016448, -335.5075075301652987 ) ) ;
#23037=CARTESIAN_POINT ( 'NONE',  ( -112.3417001280820386, -272.5521521680024648, -270.3611179825637691 ) ) ;
#23039=CARTESIAN_POINT ( 'NONE',  ( -39.11133947780892584, -293.5538666671052965, -346.6472643746234894 ) ) ;
#23040=CARTESIAN_POINT ( 'NONE',  ( 11.65007981682876981, -288.3453612610721279, -215.0996671610036799 ) ) ;
#23041=CARTESIAN_POINT ( 'NONE',  ( -108.5166941645621250, -289.1347622914310023, -243.6012486297789508 ) ) ;
#23042=CARTESIAN_POINT ( 'NONE',  ( -68.99511371268030757, -290.9020949972578478, -336.7948167171654745 ) ) ;
#23044=CARTESIAN_POINT ( 'NONE',  ( -15.79435479331285208, -289.5691331498177874, -340.3305388770136801 ) ) ;
#23045=CARTESIAN_POINT ( 'NONE',  ( -41.82201281398626946, -297.0880962903817135, -345.6342887277464229 ) ) ;
#23047=CARTESIAN_POINT ( 'NONE',  ( -3.223725644451214123, -289.8167228735741787, -338.9611848770142046 ) ) ;
#23048=CARTESIAN_POINT ( 'NONE',  ( -66.69793324462361284, -277.6895848197020200, -200.9592564668876662 ) ) ;
#23049=CARTESIAN_POINT ( 'NONE',  ( -69.95728058527336657, -279.9675463629112642, -200.6189171856417772 ) ) ;
#23050=CARTESIAN_POINT ( 'NONE',  ( -56.54727495883272326, -279.4780139250356683, -195.7615820074706221 ) ) ;
#23051=CARTESIAN_POINT ( 'NONE',  ( -41.40653712575242196, -284.0008302512565592, -195.4585063752245162 ) ) ;
#23053=CARTESIAN_POINT ( 'NONE',  ( -46.58719455689786315, -278.0732848876314733, -196.6519309690943658 ) ) ;
#23054=CARTESIAN_POINT ( 'NONE',  ( -35.96220590900719571, -281.0347259771733661, -345.3612111458625691 ) ) ;
#23056=CARTESIAN_POINT ( 'NONE',  ( -113.3514020704284491, -277.1241618676822895, -263.0608265157525238 ) ) ;
#23057=CARTESIAN_POINT ( 'NONE',  ( -103.7445085002272549, -274.4029410594257570, -238.6429535384267808 ) ) ;
#23058=CARTESIAN_POINT ( 'NONE',  ( -92.22217477566852040, -282.7347260208776447, -323.9300083195294064 ) ) ;
#23059=CARTESIAN_POINT ( 'NONE',  ( -51.60292306502575599, -274.6680237183493887, -198.5511518752886957 ) ) ;
#23060=CARTESIAN_POINT ( 'NONE',  ( -102.2283298552442119, -274.5093765130136489, -230.0085273007811963 ) ) ;
#23061=CARTESIAN_POINT ( 'NONE',  ( 29.17177926537851462, -275.6248953327231561, -300.4948954698955959 ) ) ;
#23062=CARTESIAN_POINT ( 'NONE',  ( -36.96048529847585939, -297.0475027606361778, -345.3729185345040946 ) ) ;
#23063=CARTESIAN_POINT ( 'NONE',  ( -100.6793905824125375, -290.1405600426522824, -314.1485245330976568 ) ) ;
#23064=CARTESIAN_POINT ( 'NONE',  ( -36.73901250372355776, -278.1395225728509217, -194.7907156090710430 ) ) ;
#23065=CARTESIAN_POINT ( 'NONE',  ( -112.6395228627787617, -290.5875780896378728, -254.1980526174594672 ) ) ;
#23066=CARTESIAN_POINT ( 'NONE',  ( -74.84666357450154806, -288.6234962447686598, -333.2788435033249357 ) ) ;
#23067=CARTESIAN_POINT ( 'NONE',  ( 30.39101023973152138, -291.1267789752083672, -238.0334972168624006 ) ) ;
#23068=ORIENTED_EDGE ( 'NONE', *, *, #14172, .T. ) ;
#23070=CARTESIAN_POINT ( 'NONE',  ( -109.2405925237924720, -289.8886904403756262, -283.3433255781566800 ) ) ;
#23072=CARTESIAN_POINT ( 'NONE',  ( 5.039754113410213066, -287.5508204977185756, -206.2928695170018614 ) ) ;
#23073=CARTESIAN_POINT ( 'NONE',  ( -109.1418805571601069, -287.0519495502701943, -270.3937649182068412 ) ) ;
#23074=CARTESIAN_POINT ( 'NONE',  ( -2.086246166839725191, -293.6556151164621724, -338.5510965693142680 ) ) ;
#23075=CARTESIAN_POINT ( 'NONE',  ( 6.655189435110066221, -283.7832082778465974, -333.0164210029108176 ) ) ;
#23076=CARTESIAN_POINT ( 'NONE',  ( -94.95574884498813617, -285.0173244828348516, -225.5120202439765649 ) ) ;
#23077=CARTESIAN_POINT ( 'NONE',  ( -1.496641101183209033, -275.8531247943793687, -206.1877254301955418 ) ) ;
#23078=CARTESIAN_POINT ( 'NONE',  ( -45.29039825565088506, -293.1733013604011830, -344.6331137995465497 ) ) ;
#23079=CARTESIAN_POINT ( 'NONE',  ( -43.50022387494253451, -272.7676887600310351, -197.1718852836665690 ) ) ;
#23082=CARTESIAN_POINT ( 'NONE',  ( -33.44015491470214130, -294.6710496593075845, -347.2541546797676233 ) ) ;
#23083=CARTESIAN_POINT ( 'NONE',  ( -55.12356286014078677, -287.7419957932046941, -198.0227959426889583 ) ) ;
#23084=CARTESIAN_POINT ( 'NONE',  ( -91.42730863239619055, -298.3836642213286723, -215.9898069624495349 ) ) ;
#23085=CARTESIAN_POINT ( 'NONE',  ( 33.48526286457929757, -287.9644541050095086, -252.2154794284144259 ) ) ;
#23086=CARTESIAN_POINT ( 'NONE',  ( -101.9056079770701615, -277.0633211618754785, -311.9830931275199646 ) ) ;
#23087=CARTESIAN_POINT ( 'NONE',  ( -22.22196106315864839, -292.8921925681279390, -194.9098735930651571 ) ) ;
#23088=CARTESIAN_POINT ( 'NONE',  ( -15.74253984827584496, -284.4681217844403704, -197.6858003489593898 ) ) ;
#23089=CARTESIAN_POINT ( 'NONE',  ( 37.06105332286537646, -293.6375546479075638, -250.5624990414058288 ) ) ;
#23091=CARTESIAN_POINT ( 'NONE',  ( -74.99414792047076617, -291.8692812635048881, -207.7370721497273678 ) ) ;
#23093=CARTESIAN_POINT ( 'NONE',  ( 185.1269714985386940, 260.3434729467832085, -151.0899229522644305 ) ) ;
#23094=CARTESIAN_POINT ( 'NONE',  ( -32.37109183951687186, -287.6338450157566058, -194.2034656106150408 ) ) ;
#23095=CARTESIAN_POINT ( 'NONE',  ( -37.37352853689063181, -280.5523547857346784, -350.3611179825600175 ) ) ;
#23096=ORIENTED_EDGE ( 'NONE', *, *, #56608, .F. ) ;
#23098=CARTESIAN_POINT ( 'NONE',  ( -40.26037179800940891, -282.0100258253328889, -343.6121072589616006 ) ) ;
#23099=CARTESIAN_POINT ( 'NONE',  ( -114.3638145849992327, -278.2033256827040191, -271.6038180778849664 ) ) ;
#23100=CARTESIAN_POINT ( 'NONE',  ( 5.963875701497209469, -282.6412053479145925, -209.3311620105461657 ) ) ;
#23101=CARTESIAN_POINT ( 'NONE',  ( 204.8862265131387232, 293.2993722356919761, -68.49257677906207675 ) ) ;
#23102=CARTESIAN_POINT ( 'NONE',  ( -87.35049715070886123, -283.9457885820980891, -212.5180243721792124 ) ) ;
#23104=CARTESIAN_POINT ( 'NONE',  ( 36.37978931252406056, -285.7243027336915020, -282.1466241914561692 ) ) ;
#23105=CARTESIAN_POINT ( 'NONE',  ( -57.81105076995320502, -275.6511065199740074, -197.3592595797459808 ) ) ;
#23106=CARTESIAN_POINT ( 'NONE',  ( -79.76887163852329365, -297.9532412756065582, -210.8806711187741598 ) ) ;
#23107=CARTESIAN_POINT ( 'NONE',  ( -55.94420165895228791, -293.9814351171912108, -341.5137210183028742 ) ) ;
#23108=CARTESIAN_POINT ( 'NONE',  ( -98.71704893602846198, -278.5855093591795821, -316.7117600353072930 ) ) ;
#23109=CARTESIAN_POINT ( 'NONE',  ( 34.16456340563001959, -275.7459637883437154, -285.0530979528506350 ) ) ;
#23110=CARTESIAN_POINT ( 'NONE',  ( -108.8832376279748928, -273.9848380210694359, -242.5869697181078664 ) ) ;
#23111=CARTESIAN_POINT ( 'NONE',  ( -67.59935648285741649, -276.3602814150734162, -340.8307337207493788 ) ) ;
#23112=CARTESIAN_POINT ( 'NONE',  ( -13.31626158348878874, -91.39965012456295312, -359.9159752949001927 ) ) ;
#23113=CARTESIAN_POINT ( 'NONE',  ( -96.53395615140642860, -275.9201402729734696, -316.4389672228826953 ) ) ;
#23114=CARTESIAN_POINT ( 'NONE',  ( -111.3930835316681396, -297.7392333357630605, -289.2553042699672687 ) ) ;
#23117=CARTESIAN_POINT ( 'NONE',  ( 201.7648208617462728, 289.3015991269851384, -82.29596988341933184 ) ) ;
#23118=CARTESIAN_POINT ( 'NONE',  ( -103.2847323722991462, -285.1986753534072250, -302.5048719639568162 ) ) ;
#23119=CARTESIAN_POINT ( 'NONE',  ( -109.7134906865551613, -286.0167569733327468, -293.5620943931781994 ) ) ;
#23120=CARTESIAN_POINT ( 'NONE',  ( 4.790877695016662940, -285.9863587247015744, -210.5602492379419743 ) ) ;
#23121=CARTESIAN_POINT ( 'NONE',  ( -91.56938560940982086, -276.2402371828815717, -320.4934276960730699 ) ) ;
#23122=CARTESIAN_POINT ( 'NONE',  ( -89.74980892215164374, -285.6611360427416457, -323.0094337614041251 ) ) ;
#23123=CARTESIAN_POINT ( 'NONE',  ( -16.70922533298621104, -278.8034489925120170, -199.6150316263843649 ) ) ;
#23124=CARTESIAN_POINT ( 'NONE',  ( -70.58071852552338044, -278.5809021355741493, -335.7017158562146619 ) ) ;
#23126=CARTESIAN_POINT ( 'NONE',  ( 9.001565720888773825, -299.2987937108537722, -197.2538927750957782 ) ) ;
#23127=CARTESIAN_POINT ( 'NONE',  ( 38.26851345264829973, -282.5273960088877061, -284.1183472288806797 ) ) ;
#23129=CARTESIAN_POINT ( 'NONE',  ( -33.05590202049050674, -283.4919033845052923, -347.1932429325181033 ) ) ;
#23133=CARTESIAN_POINT ( 'NONE',  ( -7.846218032262715525, -288.2948082872201780, -200.5176880699377193 ) ) ;
#23134=CARTESIAN_POINT ( 'NONE',  ( -82.57464792869529902, -288.3407322873807175, -332.0642678598034081 ) ) ;
#23135=CARTESIAN_POINT ( 'NONE',  ( -109.8950036751649861, -295.8782574299456769, -260.5650054114635168 ) ) ;
#23137=CARTESIAN_POINT ( 'NONE',  ( 23.03320857062457350, -292.2627004819572676, -222.7146264494023171 ) ) ;
#23138=CARTESIAN_POINT ( 'NONE',  ( 22.51363516826799227, -286.6273581318101265, -313.3500303904747852 ) ) ;
#23139=CARTESIAN_POINT ( 'NONE',  ( -10.52616955324940484, -287.2701896116669218, -338.9453373976196531 ) ) ;
#23140=CARTESIAN_POINT ( 'NONE',  ( -30.69394174215420534, -290.3771977414566550, -196.6469312759338663 ) ) ;
#23141=CARTESIAN_POINT ( 'NONE',  ( -70.17374683063228247, -286.8146969797601855, -204.7026970882218677 ) ) ;
#23142=CARTESIAN_POINT ( 'NONE',  ( -104.5643897065728680, -276.1118192978071875, -303.7362850233948848 ) ) ;
#23143=CARTESIAN_POINT ( 'NONE',  ( 21.77149474858413569, -286.6041409881937625, -318.4656412901785529 ) ) ;
#23144=CARTESIAN_POINT ( 'NONE',  ( 36.98962690132006514, -289.4240087407114288, -260.3683971037505671 ) ) ;
#23145=CARTESIAN_POINT ( 'NONE',  ( -79.53313586798829249, -287.6200394206268811, -332.6326208329983274 ) ) ;
#23146=CARTESIAN_POINT ( 'NONE',  ( -78.49899755629139975, -284.5627539808037341, -330.9373948245737438 ) ) ;
#23147=CARTESIAN_POINT ( 'NONE',  ( -96.04806698317332803, -293.1963925878686723, -223.4186966317512031 ) ) ;
#23150=CARTESIAN_POINT ( 'NONE',  ( -82.13692737016141621, -299.3671430803469207, -209.4462635934506238 ) ) ;
#23151=CARTESIAN_POINT ( 'NONE',  ( 31.22521321643745651, -280.4079841052864595, -244.6974888225194320 ) ) ;
#23152=CARTESIAN_POINT ( 'NONE',  ( 22.95158276074157655, -278.9430459095565880, -225.7332082813008753 ) ) ;
#23153=CARTESIAN_POINT ( 'NONE',  ( 37.90586491131076485, -292.5535674558253731, -254.7414366649772717 ) ) ;
#23154=CARTESIAN_POINT ( 'NONE',  ( -91.85391228343023329, -271.5009101324063181, -220.2784769973490597 ) ) ;
#23155=CARTESIAN_POINT ( 'NONE',  ( 20.28104307434243481, -274.2866120228680415, -317.5079784737774844 ) ) ;
#23156=CARTESIAN_POINT ( 'NONE',  ( -106.4451965586153932, -297.5345032664055793, -295.5296603855035187 ) ) ;
#23157=DIRECTION ( 'NONE',  ( 1.000000000000000000, 0.000000000000000000, 0.000000000000000000 ) ) ;
#23158=CARTESIAN_POINT ( 'NONE',  ( -63.33942902849123868, -272.2946685124165356, -198.5090172173570409 ) ) ;
#23159=CARTESIAN_POINT ( 'NONE',  ( -112.2094488735885420, -294.6235898437623177, -283.6510303108961466 ) ) ;
#23161=CARTESIAN_POINT ( 'NONE',  ( 34.02188085833573439, -295.2125768825517298, -288.3225830535881187 ) ) ;
#23163=CARTESIAN_POINT ( 'NONE',  ( -78.03107744932488288, -296.4170835911325526, -331.2250690876712724 ) ) ;
#23164=PLANE ( 'NONE',  #39921 ) ;
#23166=CARTESIAN_POINT ( 'NONE',  ( -67.81205731565275130, -283.6743745887989121, -201.4270676777732376 ) ) ;
#23167=CARTESIAN_POINT ( 'NONE',  ( -79.72804649810302635, -297.4609733392965722, -210.9271408196563868 ) ) ;
#23169=CARTESIAN_POINT ( 'NONE',  ( -74.27598446526295106, -283.5288494502705703, -337.9843474849482163 ) ) ;
#23170=CARTESIAN_POINT ( 'NONE',  ( 38.18129690616638072, -283.5024435202262225, -272.7256716900491824 ) ) ;
#23171=CARTESIAN_POINT ( 'NONE',  ( -80.92273809564112241, -285.1451956848103464, -206.8425642336146097 ) ) ;
#23172=CARTESIAN_POINT ( 'NONE',  ( -1.540488127866042944, -290.5276815231948717, -204.6327781894834459 ) ) ;
#23173=CARTESIAN_POINT ( 'NONE',  ( 10.59707575819633618, -273.9094976428775681, -330.5268031993606428 ) ) ;
#23176=CARTESIAN_POINT ( 'NONE',  ( 13.49267389295802744, -285.4664077818697479, -217.2144373099860104 ) ) ;
#23177=CARTESIAN_POINT ( 'NONE',  ( -112.8652126534752540, -289.6398681779726871, -257.0310179803962569 ) ) ;
#23179=CARTESIAN_POINT ( 'NONE',  ( -99.12839207723251889, -298.7066111322874917, -229.9096502077262016 ) ) ;
#23180=CARTESIAN_POINT ( 'NONE',  ( -90.66011675739846964, -280.7398643825711133, -215.5538671777336219 ) ) ;
#23181=CARTESIAN_POINT ( 'NONE',  ( 22.70276846251368497, -292.1921377247896316, -315.8920810494681746 ) ) ;
#23182=CARTESIAN_POINT ( 'NONE',  ( 30.04263589383815258, -280.8416039714027761, -242.2285968445845299 ) ) ;
#23183=CARTESIAN_POINT ( 'NONE',  ( -72.07213583812325908, -295.6654071016297962, -339.0837259068874801 ) ) ;
#23185=CARTESIAN_POINT ( 'NONE',  ( -32.37616501558099458, -284.1941243810745732, -194.9515292680658547 ) ) ;
#23186=CARTESIAN_POINT ( 'NONE',  ( -87.61032342335124667, -281.3504217482249032, -214.7008434753115864 ) ) ;
#23187=CARTESIAN_POINT ( 'NONE',  ( -68.62871233428695916, -294.5324232815688106, -336.5906878928592505 ) ) ;
#23188=CARTESIAN_POINT ( 'NONE',  ( -37.23030460611856540, -296.0533920991546779, -195.3604033763125187 ) ) ;
#23192=CARTESIAN_POINT ( 'NONE',  ( 32.91099910132031425, -283.8623807971577548, -295.7411597350413786 ) ) ;
#23193=CARTESIAN_POINT ( 'NONE',  ( -95.65723462145159317, -295.4417982783928096, -314.3963507363878307 ) ) ;
#23195=CARTESIAN_POINT ( 'NONE',  ( -4.829096099716524648, -280.1237833571632336, -337.9475929042657754 ) ) ;
#23196=CARTESIAN_POINT ( 'NONE',  ( -73.85908977557677701, -272.7773911846299484, -202.6954716124624269 ) ) ;
#23197=CARTESIAN_POINT ( 'NONE',  ( -92.41312301962470599, -289.7015755172369040, -318.3546998379551383 ) ) ;
#23198=CARTESIAN_POINT ( 'NONE',  ( -62.56427261639770165, -281.2381611747639454, -201.0647058391529072 ) ) ;
#23199=CARTESIAN_POINT ( 'NONE',  ( -67.40181763168531859, -275.2513320519411195, -202.9467554711895616 ) ) ;
#23200=VECTOR ( 'NONE', #6684, 1000.000000000000000 ) ;
#23201=CARTESIAN_POINT ( 'NONE',  ( 21.01066939769183506, -283.8189942461900159, -319.3656217377672419 ) ) ;
#23202=CARTESIAN_POINT ( 'NONE',  ( -11.58953084956374369, -279.1899416906577471, -201.5763216191979836 ) ) ;
#23203=CARTESIAN_POINT ( 'NONE',  ( 10.97131902505812562, -278.3837087079525645, -327.7270732700507665 ) ) ;
#23205=CARTESIAN_POINT ( 'NONE',  ( -68.84212266237791766, -273.4826822037952638, -200.0849027925046926 ) ) ;
#23206=CARTESIAN_POINT ( 'NONE',  ( -17.06335767002813952, -294.2360154427400403, -198.6827564499790526 ) ) ;
#23210=CARTESIAN_POINT ( 'NONE',  ( -63.85646719829682638, -293.5338488162076374, -341.3348638840794251 ) ) ;
#23211=CARTESIAN_POINT ( 'NONE',  ( -66.82398576107701160, -297.3216081865396632, -203.5426269840474731 ) ) ;
#23213=CARTESIAN_POINT ( 'NONE',  ( -66.76613668881105923, -293.1936707411405223, -199.9557894442065447 ) ) ;
#23214=CARTESIAN_POINT ( 'NONE',  ( -95.95921662488163406, -280.4090924074130839, -317.1477375740089997 ) ) ;
#23215=CARTESIAN_POINT ( 'NONE',  ( 37.48866874839452379, -289.5608954803890356, -271.0276891956934264 ) ) ;
#23216=CARTESIAN_POINT ( 'NONE',  ( 1.809409478635427559, -274.5274096658723124, -334.1967465040609682 ) ) ;
#23217=CARTESIAN_POINT ( 'NONE',  ( 31.62113498613430096, -277.8420504543230436, -298.5241164368026716 ) ) ;
#23218=CARTESIAN_POINT ( 'NONE',  ( 9.108005016690839284, -292.4890540038915674, -328.5972628349492197 ) ) ;
#23219=CARTESIAN_POINT ( 'NONE',  ( -110.8926297111280519, -280.6443336381020686, -252.1263398958670905 ) ) ;
#23221=CARTESIAN_POINT ( 'NONE',  ( -82.81120301710156184, -283.3602070823393433, -327.5627857347354279 ) ) ;
#23222=CARTESIAN_POINT ( 'NONE',  ( -101.6395985165605680, -280.1840719848489698, -228.4646074202884733 ) ) ;
#23224=CARTESIAN_POINT ( 'NONE',  ( -70.31319262419275162, -282.2719379550259191, -339.5194819836434021 ) ) ;
#23225=CARTESIAN_POINT ( 'NONE',  ( -86.93402125105039602, -278.6638060523109175, -329.0260674517909365 ) ) ;
#23226=CARTESIAN_POINT ( 'NONE',  ( 5.498173904724613870, -278.0035894714825986, -333.5074000915728334 ) ) ;
#23227=CARTESIAN_POINT ( 'NONE',  ( -67.68488546085839630, -291.9805209788416391, -333.4427485647536855 ) ) ;
#23229=CARTESIAN_POINT ( 'NONE',  ( -110.1217768095011991, -298.7855627655889634, -252.1960095164200197 ) ) ;
#23231=CARTESIAN_POINT ( 'NONE',  ( -60.36905172503362849, -292.8262349178734212, -200.7092348225381215 ) ) ;
#23232=CARTESIAN_POINT ( 'NONE',  ( -71.22137473659145712, -275.5218334964210953, -336.8743832344716793 ) ) ;
#23233=CARTESIAN_POINT ( 'NONE',  ( -6.023395597853273387, -290.4062899862208837, -339.5936090380857308 ) ) ;
#23234=CARTESIAN_POINT ( 'NONE',  ( -89.88382808080551456, -290.6341816295014269, -219.5357556290681487 ) ) ;
#23235=CARTESIAN_POINT ( 'NONE',  ( 39.29397142541546373, -286.9672888522335370, -262.9694154054036517 ) ) ;
#23237=CARTESIAN_POINT ( 'NONE',  ( -51.18775407657944498, -281.6318124543672070, -342.9027590173910767 ) ) ;
#23238=CARTESIAN_POINT ( 'NONE',  ( -71.72415620242954049, -291.3718850251189565, -336.1684269271525523 ) ) ;
#23239=CARTESIAN_POINT ( 'NONE',  ( -110.6824360606842959, -283.1326777471875857, -262.6585213728271242 ) ) ;
#23240=CARTESIAN_POINT ( 'NONE',  ( -22.10843189992635871, -281.5664342479233824, -198.4118262717569223 ) ) ;
#23242=CARTESIAN_POINT ( 'NONE',  ( -104.9430788388014975, -291.0216986242278949, -306.7324502201704490 ) ) ;
#23243=TOROIDAL_SURFACE ( 'NONE', #68604, 5.654241149514406040, 1.000000000000000000 ) ;
#23244=CARTESIAN_POINT ( 'NONE',  ( -108.8236835104323319, -278.8453416376117389, -285.4711971875941572 ) ) ;
#23245=CARTESIAN_POINT ( 'NONE',  ( 30.55413562263701266, -291.8857969571606645, -234.7762722596812353 ) ) ;
#23246=CARTESIAN_POINT ( 'NONE',  ( 25.40731789069867474, -287.7666116624911865, -225.9907249690027413 ) ) ;
#23247=CARTESIAN_POINT ( 'NONE',  ( -12.23787821491825412, -289.2265948227954482, -343.1446926993477859 ) ) ;
#23248=CARTESIAN_POINT ( 'NONE',  ( -46.72697293178587330, -286.0965006771618846, -197.9161668777973944 ) ) ;
#23251=CARTESIAN_POINT ( 'NONE',  ( -11.59563683910588416, -294.2441977125491235, -199.0497891597565570 ) ) ;
#23252=AXIS2_PLACEMENT_3D ( 'NONE', #77796, #91506, #77318 ) ;
#23253=CARTESIAN_POINT ( 'NONE',  ( -107.9265843327669216, -294.8576346342608758, -300.0122397331491015 ) ) ;
#23254=CONICAL_SURFACE ( 'NONE', #15693, 2.241321557046427326, 0.09862129276975473147 ) ;
#23255=CARTESIAN_POINT ( 'NONE',  ( -48.65598010146408825, -276.2583610780988579, -342.7687068352769870 ) ) ;
#23256=CARTESIAN_POINT ( 'NONE',  ( -109.7520853079921608, -296.2279283463375918, -244.4758151155552071 ) ) ;
#23257=CARTESIAN_POINT ( 'NONE',  ( 34.32654477548992134, -291.8071658631701553, -253.1499209683281606 ) ) ;
#23258=CARTESIAN_POINT ( 'NONE',  ( -104.8702353662897906, -294.3880289069327887, -300.7828693776153273 ) ) ;
#23259=CARTESIAN_POINT ( 'NONE',  ( -65.49337432703740092, -292.8807851693272823, -202.5639486850024298 ) ) ;
#23260=CARTESIAN_POINT ( 'NONE',  ( 16.39504089865694425, -295.3454948886044349, -320.2268250129523608 ) ) ;
#23261=CARTESIAN_POINT ( 'NONE',  ( 145.2857639756989272, -299.5541904835127980, -201.0153591320744226 ) ) ;
#23262=CARTESIAN_POINT ( 'NONE',  ( -55.64901225581454725, -293.2871030229669032, -343.2642780386795494 ) ) ;
#23263=CARTESIAN_POINT ( 'NONE',  ( -94.36988634794697361, -299.2270841038119329, -221.6305095276072450 ) ) ;
#23264=CARTESIAN_POINT ( 'NONE',  ( -101.8447249312820446, -291.0207030784135327, -305.1495542590761829 ) ) ;
#23265=CARTESIAN_POINT ( 'NONE',  ( -20.83927121544913774, -295.1678696842265595, -341.5452097418858557 ) ) ;
#23266=CARTESIAN_POINT ( 'NONE',  ( -73.28952984851748909, -279.5062559411719576, -336.6038905178002096 ) ) ;
#23267=CARTESIAN_POINT ( 'NONE',  ( -38.14780144950937313, -278.7270804416718875, -193.8585136119885703 ) ) ;
#23269=EDGE_CURVE ( 'NONE', #29794, #43403, #91127, .T. ) ;
#23270=CARTESIAN_POINT ( 'NONE',  ( -36.93193448223406961, -273.4057789934512357, -193.4511072721188043 ) ) ;
#23271=CARTESIAN_POINT ( 'NONE',  ( 34.50981191351140609, -279.3793453141463488, -250.8527308020481712 ) ) ;
#23272=CARTESIAN_POINT ( 'NONE',  ( -111.9302186717079763, -277.1498190171853935, -254.7100334137157915 ) ) ;
#23273=CARTESIAN_POINT ( 'NONE',  ( -109.5683945903965224, -276.8193602342198574, -249.5444651516260990 ) ) ;
#23275=CARTESIAN_POINT ( 'NONE',  ( -37.13149631189084943, -296.7396699976850982, -196.8651434942196090 ) ) ;
#23277=CARTESIAN_POINT ( 'NONE',  ( -109.2207238160707163, -288.2797955091778022, -293.1550527246924958 ) ) ;
#23278=CARTESIAN_POINT ( 'NONE',  ( -85.16467598022127561, -289.6915113693370927, -330.7778249780870397 ) ) ;
#23280=CARTESIAN_POINT ( 'NONE',  ( -65.56310310867200997, -275.6841838584450670, -200.6796372794978254 ) ) ;
#23281=CARTESIAN_POINT ( 'NONE',  ( -80.77184926015803512, -295.4611348635506829, -209.4197480422085391 ) ) ;
#23282=CARTESIAN_POINT ( 'NONE',  ( -34.49521044067520137, -282.2143964689399809, -347.1468999825981427 ) ) ;
#23285=CARTESIAN_POINT ( 'NONE',  ( 37.56699174476693059, -279.4925984755161608, -265.7357445968982006 ) ) ;
#23287=CARTESIAN_POINT ( 'NONE',  ( 11.20487646469172915, -291.5370370169802072, -215.2445762560115554 ) ) ;
#23288=CARTESIAN_POINT ( 'NONE',  ( -110.1356125781775575, -282.8805732588281217, -255.8039275575864622 ) ) ;
#23291=CARTESIAN_POINT ( 'NONE',  ( 25.01795185599723581, -290.9887891369123736, -228.6924912560687062 ) ) ;
#23292=CARTESIAN_POINT ( 'NONE',  ( -62.03855187148693773, -278.9786648920089078, -339.9604337565301080 ) ) ;
#23293=CARTESIAN_POINT ( 'NONE',  ( 15.49083027676914526, -283.5298621676657262, -325.8294192801051850 ) ) ;
#23294=CARTESIAN_POINT ( 'NONE',  ( -91.12656288406512317, -271.3749277186235531, -217.2903846593624166 ) ) ;
#23295=CARTESIAN_POINT ( 'NONE',  ( -83.64786928081187511, -285.3964072233478646, -213.8619499687001735 ) ) ;
#23296=CARTESIAN_POINT ( 'NONE',  ( 14.15653979063705314, -277.7371666531194023, -322.9992634733325758 ) ) ;
#23297=CARTESIAN_POINT ( 'NONE',  ( -48.62267331036382245, -278.0021648618229619, -342.6991424076827002 ) ) ;
#23298=CARTESIAN_POINT ( 'NONE',  ( -89.04056962133726927, -285.7786127781236019, -324.7667082790004542 ) ) ;
#23302=CARTESIAN_POINT ( 'NONE',  ( -111.2159886395630650, -296.1125483779802607, -292.1237406227365909 ) ) ;
#23303=CARTESIAN_POINT ( 'NONE',  ( 27.79052400944419787, -289.0429914653246897, -233.7911935675299446 ) ) ;
#23305=CARTESIAN_POINT ( 'NONE',  ( -115.3430155898818299, -287.8380690714489560, -288.1317622949166548 ) ) ;
#23306=CARTESIAN_POINT ( 'NONE',  ( -97.44603533916775007, -278.1124905655667021, -222.7275016991840744 ) ) ;
#23307=CARTESIAN_POINT ( 'NONE',  ( -27.92750716894570218, -290.5695084754560185, -194.6917755602924274 ) ) ;
#23310=CARTESIAN_POINT ( 'NONE',  ( -105.8514168628970111, -285.7108616742070808, -297.6500058103541733 ) ) ;
#23311=CARTESIAN_POINT ( 'NONE',  ( -90.21293732324741654, -281.0523667242918009, -218.4945783500481582 ) ) ;
#23312=CARTESIAN_POINT ( 'NONE',  ( 30.88744572837336122, -288.5313313166724356, -235.9606827091901948 ) ) ;
#23313=CARTESIAN_POINT ( 'NONE',  ( 20.92141384490246736, -284.2028694481392677, -317.6085879122549045 ) ) ;
#23314=CARTESIAN_POINT ( 'NONE',  ( 19.87862433691756792, -276.4184067058993151, -321.9059365171859213 ) ) ;
#23315=CARTESIAN_POINT ( 'NONE',  ( 54.21872727873468278, -297.2238285168403422, -195.7474017060856113 ) ) ;
#23316=CARTESIAN_POINT ( 'NONE',  ( -48.11668167676107544, -279.7521365748772837, -194.0648984730356688 ) ) ;
#23318=CARTESIAN_POINT ( 'NONE',  ( -60.99620677641041766, -299.6630280932378696, -199.7248724386597587 ) ) ;
#23322=CARTESIAN_POINT ( 'NONE',  ( -55.07509983363680561, -272.0669901721399242, -196.4726848811926629 ) ) ;
#23323=CARTESIAN_POINT ( 'NONE',  ( 129.9467878515196162, -299.5541904835127980, -195.3611179825600175 ) ) ;
#23324=CARTESIAN_POINT ( 'NONE',  ( -16.89849494288845833, -279.8310582924833625, -200.2179515067299462 ) ) ;
#23326=CARTESIAN_POINT ( 'NONE',  ( -63.43632891748307401, -274.9245924192893540, -198.3397387500548064 ) ) ;
#23327=CARTESIAN_POINT ( 'NONE',  ( 37.10600378377182551, -280.3759911695543678, -251.6432229072009363 ) ) ;
#23328=CARTESIAN_POINT ( 'NONE',  ( -74.02803292616864894, -291.3067595809320096, -334.6570387889773883 ) ) ;
#23329=CARTESIAN_POINT ( 'NONE',  ( -59.96120240422219183, -299.2844946955736418, -197.4290307838639364 ) ) ;
#23331=CARTESIAN_POINT ( 'NONE',  ( -87.21543557016718751, -298.5804568805023678, -212.1480869423973843 ) ) ;
#23332=CARTESIAN_POINT ( 'NONE',  ( -32.05250701161843807, -294.1191701809748906, -195.7019962100786188 ) ) ;
#23333=CARTESIAN_POINT ( 'NONE',  ( 29.42842234223097364, -279.1031206889799705, -236.4559201851825776 ) ) ;
#23334=CARTESIAN_POINT ( 'NONE',  ( 35.46864646699807366, -283.2711528789251361, -254.8095909193533544 ) ) ;
#23335=CARTESIAN_POINT ( 'NONE',  ( -84.20405779875382279, -271.4240705508181009, -212.2597734791546031 ) ) ;
#23336=CARTESIAN_POINT ( 'NONE',  ( -113.1062432911641338, -286.0494738921869384, -278.4958837259513871 ) ) ;
#23338=CARTESIAN_POINT ( 'NONE',  ( 8.161102698606372385, -287.3330513106757849, -327.8391225368562232 ) ) ;
#23339=CARTESIAN_POINT ( 'NONE',  ( -112.2160709410385238, -274.3727637374173582, -284.1527603578829257 ) ) ;
#23341=CARTESIAN_POINT ( 'NONE',  ( -12.43309089404968582, -287.3092843456158221, -342.6534409828449270 ) ) ;
#23342=CARTESIAN_POINT ( 'NONE',  ( -82.56268449359332351, -289.3565593180966857, -327.6947909827397325 ) ) ;
#23344=CARTESIAN_POINT ( 'NONE',  ( -32.34036460503271115, -287.1934655579176479, -193.8203679819181104 ) ) ;
#23345=CARTESIAN_POINT ( 'NONE',  ( 20.69575246798601853, -275.2621750811438233, -226.0264138379587848 ) ) ;
#23346=CARTESIAN_POINT ( 'NONE',  ( 37.46286475800634719, -292.2595500284507466, -253.3974698893223660 ) ) ;
#23347=CARTESIAN_POINT ( 'NONE',  ( 37.23037318310591814, -281.9683987575965034, -251.5909643053241211 ) ) ;
#23348=CARTESIAN_POINT ( 'NONE',  ( 36.31067086039960401, -282.8195813053796428, -250.3607749432480887 ) ) ;
#23349=CARTESIAN_POINT ( 'NONE',  ( -86.08570385405211312, -284.0403258403158020, -329.9410339962473131 ) ) ;
#23351=CARTESIAN_POINT ( 'NONE',  ( -16.91986785000901250, -280.6565537443357812, -200.2537984424178603 ) ) ;
#23352=CARTESIAN_POINT ( 'NONE',  ( -92.05005921254146983, -294.6952119285919025, -226.6919474004047572 ) ) ;
#23353=CARTESIAN_POINT ( 'NONE',  ( 198.0283610688475733, 285.1170005366674900, -111.8712284615754413 ) ) ;
#23355=CARTESIAN_POINT ( 'NONE',  ( -94.10095716986310777, -279.8749314876756671, -319.1301160161154939 ) ) ;
#23356=CARTESIAN_POINT ( 'NONE',  ( -57.10806838110030981, -168.8649533382279060, -363.8072750875188035 ) ) ;
#23357=CARTESIAN_POINT ( 'NONE',  ( -86.16221177476658966, -296.7019530828766278, -215.9510976696027171 ) ) ;
#23358=CARTESIAN_POINT ( 'NONE',  ( 23.93002802275086438, -292.4389926912623423, -223.8066277808137272 ) ) ;
#23359=CARTESIAN_POINT ( 'NONE',  ( -29.93913374795647542, -125.2961201611392568, -360.6981843052933527 ) ) ;
#23360=CARTESIAN_POINT ( 'NONE',  ( -26.29730116933454553, -296.7626041866188302, -193.9529577754875902 ) ) ;
#23361=CARTESIAN_POINT ( 'NONE',  ( -99.52671033333007244, -288.4082832812932224, -310.1036005480806921 ) ) ;
#23362=CARTESIAN_POINT ( 'NONE',  ( -7.469891723505769576, -296.5167088783151712, -338.3347726063263963 ) ) ;
#23363=CARTESIAN_POINT ( 'NONE',  ( -52.20492163588632906, -287.1730334191447014, -198.3866216452606182 ) ) ;
#23365=CARTESIAN_POINT ( 'NONE',  ( -4.592002640016518811, -295.5724248616011778, -339.8037634367398141 ) ) ;
#23366=CARTESIAN_POINT ( 'NONE',  ( -94.17386315521936524, -285.6934710643051858, -224.4273059376094750 ) ) ;
#23367=CARTESIAN_POINT ( 'NONE',  ( -36.17639422181220255, -296.8613671933729847, -193.7584200153915788 ) ) ;
#23368=CARTESIAN_POINT ( 'NONE',  ( 8.745887779062593737, -293.4684845264431488, -208.8122564151247502 ) ) ;
#23369=CARTESIAN_POINT ( 'NONE',  ( 36.31260720565570210, -294.3258991373899107, -292.7805723015426338 ) ) ;
#23370=CARTESIAN_POINT ( 'NONE',  ( -109.9731005101578631, -290.8154837541315487, -263.0344759800364614 ) ) ;
#23373=CARTESIAN_POINT ( 'NONE',  ( -84.46694427061599697, -299.2715530945168325, -211.0356020364245353 ) ) ;
#23374=CARTESIAN_POINT ( 'NONE',  ( -10.47243879690600288, -273.1898464362398045, -198.5686975274963402 ) ) ;
#23376=CARTESIAN_POINT ( 'NONE',  ( 20.76964992338365690, -275.7419473887630375, -320.8052354438478346 ) ) ;
#23377=CARTESIAN_POINT ( 'NONE',  ( -39.16627194019173430, -296.5087532886450390, -196.6778457893443601 ) ) ;
#23378=CARTESIAN_POINT ( 'NONE',  ( -57.47051235682460657, -281.6499796111602905, -198.9069620776855629 ) ) ;
#23379=CARTESIAN_POINT ( 'NONE',  ( 17.42670940123061740, -274.3988775921335446, -320.4928113953597517 ) ) ;
#23380=CARTESIAN_POINT ( 'NONE',  ( -94.02612215519287986, -274.2877440152159352, -223.8538272194856802 ) ) ;
#23381=CARTESIAN_POINT ( 'NONE',  ( -90.37523738873673551, -274.2195596235882249, -219.8368037000986703 ) ) ;
#23382=CARTESIAN_POINT ( 'NONE',  ( 74.89888025017330619, -301.0353604444513849, -194.1311006668066739 ) ) ;
#23383=CARTESIAN_POINT ( 'NONE',  ( -34.14713859778311900, -272.1122560616433361, -195.0736583253548417 ) ) ;
#23384=CARTESIAN_POINT ( 'NONE',  ( -34.28864567643706351, -295.6641704521555880, -343.3992691567017914 ) ) ;
#23385=CARTESIAN_POINT ( 'NONE',  ( 36.21083636208848588, -292.0964652252480391, -268.0374804507874842 ) ) ;
#23387=CARTESIAN_POINT ( 'NONE',  ( -54.11172239103611048, -277.7541360401057204, -345.5042831394254108 ) ) ;
#23388=CARTESIAN_POINT ( 'NONE',  ( -1.724484571943819766, -274.7048162735077312, -206.6254271636781823 ) ) ;
#23391=CARTESIAN_POINT ( 'NONE',  ( -103.9956589051564890, -282.7452900616530087, -308.0257229134611521 ) ) ;
#23392=CARTESIAN_POINT ( 'NONE',  ( -108.5994234780850292, -298.2436910453701557, -294.2852749985610217 ) ) ;
#23395=CARTESIAN_POINT ( 'NONE',  ( -79.39376050813815766, -284.6655375083424246, -210.4305239951248154 ) ) ;
#23397=CARTESIAN_POINT ( 'NONE',  ( -68.45150373048697645, -281.4597367707630724, -338.8018569790756942 ) ) ;
#23398=CARTESIAN_POINT ( 'NONE',  ( -107.3966977611688094, -277.1068782013626901, -246.3235212932698630 ) ) ;
#23399=CARTESIAN_POINT ( 'NONE',  ( -48.71668498755099819, -275.7744186996101234, -343.1177008166039855 ) ) ;
#23400=CARTESIAN_POINT ( 'NONE',  ( 30.85635034804982979, -283.1412119372277516, -239.0284951441596490 ) ) ;
#23401=CARTESIAN_POINT ( 'NONE',  ( 29.52227771575282489, -277.1630046710104125, -300.6322093164892522 ) ) ;
#23403=CARTESIAN_POINT ( 'NONE',  ( 32.28048319347293216, -274.3514764125042689, -301.3319430120811262 ) ) ;
#23404=CARTESIAN_POINT ( 'NONE',  ( -40.94657607603063809, -282.0070757796791554, -195.2680576550856983 ) ) ;
#23406=CARTESIAN_POINT ( 'NONE',  ( -37.99499693586979987, -287.9641754973689558, -194.8039382734148148 ) ) ;
#23407=CARTESIAN_POINT ( 'NONE',  ( -110.2140130185359368, -271.2396475792842807, -270.3444066551136871 ) ) ;
#23408=CARTESIAN_POINT ( 'NONE',  ( -53.68086286175488908, -289.8424574493982391, -197.1099487432183821 ) ) ;
#23411=CARTESIAN_POINT ( 'NONE',  ( -79.94613302176524883, -296.2560916027570670, -210.5949670137222824 ) ) ;
#23412=CARTESIAN_POINT ( 'NONE',  ( -109.9131720686559390, -288.8944701100449493, -254.7327161467352141 ) ) ;
#23413=CARTESIAN_POINT ( 'NONE',  ( 2.709286185474054420, -58.23210827017373248, -348.3322198635470954 ) ) ;
#23414=CARTESIAN_POINT ( 'NONE',  ( 10.54962298731482839, -296.6514948947842640, -195.3774371216965164 ) ) ;
#23415=CARTESIAN_POINT ( 'NONE',  ( 16.18567835318193460, -286.7895243775723202, -324.8177292032018499 ) ) ;
#23416=CARTESIAN_POINT ( 'NONE',  ( -51.14779310791936950, -284.8315542291692850, -342.9103760623195285 ) ) ;
#23417=CARTESIAN_POINT ( 'NONE',  ( -62.84001718050091512, -283.9645456850599317, -198.7803255844399075 ) ) ;
#23418=CARTESIAN_POINT ( 'NONE',  ( -109.2767602435404228, -290.7198480589157725, -257.6488530210459089 ) ) ;
#23419=CARTESIAN_POINT ( 'NONE',  ( 25.63118785651181142, -282.4563228996513544, -232.1862957384384174 ) ) ;
#23420=CARTESIAN_POINT ( 'NONE',  ( 7.901823547758239030, -283.2189089445976151, -327.9203933308711498 ) ) ;
#23421=CARTESIAN_POINT ( 'NONE',  ( -8.831554727571921504, -290.6609471553683193, -340.1287799265948593 ) ) ;
#23422=CARTESIAN_POINT ( 'NONE',  ( -40.44238317311387476, -298.1809966196762502, -193.3714470020651106 ) ) ;
#23423=CARTESIAN_POINT ( 'NONE',  ( -8.800162087940272215, -286.7615306336245453, -340.3372107325507159 ) ) ;
#23424=CARTESIAN_POINT ( 'NONE',  ( -2.557543758611196871, -274.4993504954848049, -201.6509825507039295 ) ) ;
#23425=CARTESIAN_POINT ( 'NONE',  ( -67.24565010694620071, -293.6379794294977046, -201.9681316400787807 ) ) ;
#23427=CARTESIAN_POINT ( 'NONE',  ( -20.19161114001083490, -285.3376638359844719, -345.3538533559490702 ) ) ;
#23428=CARTESIAN_POINT ( 'NONE',  ( -111.8952730818596280, -276.6797949464923931, -260.3853060289647487 ) ) ;
#23430=CARTESIAN_POINT ( 'NONE',  ( -75.36287091201697308, -295.9543105265284453, -204.2639812833216695 ) ) ;
#23431=CARTESIAN_POINT ( 'NONE',  ( 19.94054786046952543, -274.2603739588362828, -224.9248247189719336 ) ) ;
#23432=CARTESIAN_POINT ( 'NONE',  ( -101.7388825753190389, -292.5587986142359114, -234.4273512581287946 ) ) ;
#23433=CARTESIAN_POINT ( 'NONE',  ( -106.7982333311414465, -291.8008097581132461, -247.1404710609513415 ) ) ;
#23434=CARTESIAN_POINT ( 'NONE',  ( -91.46742973379453190, -285.5962275565122468, -320.8425938768648393 ) ) ;
#23435=CARTESIAN_POINT ( 'NONE',  ( 22.63419704107917596, -294.3390496182859692, -222.9957548681978778 ) ) ;
#23436=CARTESIAN_POINT ( 'NONE',  ( 19.04083200773630224, -294.1591926123075496, -218.6474027522131678 ) ) ;
#23437=CARTESIAN_POINT ( 'NONE',  ( 25.79159982292571485, -293.8882793100639219, -307.0106260527365407 ) ) ;
#23438=CARTESIAN_POINT ( 'NONE',  ( 36.97445196070918882, -289.4177090016124225, -259.8777638137207759 ) ) ;
#23439=CARTESIAN_POINT ( 'NONE',  ( 25.93153829849026337, -282.2987629140076251, -314.2647969230076797 ) ) ;
#23440=CARTESIAN_POINT ( 'NONE',  ( -70.08253734947092539, -295.7040313650891790, -202.2630138902113970 ) ) ;
#23441=CARTESIAN_POINT ( 'NONE',  ( -71.06431610092320739, -285.4526513453951679, -201.1383964491991776 ) ) ;
#23442=CARTESIAN_POINT ( 'NONE',  ( 34.48735205319458430, -277.7951493866578403, -290.7164237667528823 ) ) ;
#23443=CARTESIAN_POINT ( 'NONE',  ( -83.88789911814953371, -284.1915253829378116, -213.5449223988324547 ) ) ;
#23444=CARTESIAN_POINT ( 'NONE',  ( 4.421944806646524562, -286.4885950570701993, -332.6571741056147857 ) ) ;
#23445=CARTESIAN_POINT ( 'NONE',  ( -58.92719763480694439, -277.9153763641402861, -197.7362477542605461 ) ) ;
#23446=CARTESIAN_POINT ( 'NONE',  ( -49.37856652629597676, -155.6656457446864010, -366.7448178265262868 ) ) ;
#23447=CARTESIAN_POINT ( 'NONE',  ( -110.0550090738036744, -284.1602869175135311, -262.7374027660993079 ) ) ;
#23448=CARTESIAN_POINT ( 'NONE',  ( 39.31301473653432765, -282.7516456136942793, -269.9171724271684525 ) ) ;
#23449=CARTESIAN_POINT ( 'NONE',  ( -106.3074097421376365, -289.1753056467402985, -304.1947568983028418 ) ) ;
#23450=CARTESIAN_POINT ( 'NONE',  ( -84.35660642430981682, -279.2866338203835994, -330.3951334378114097 ) ) ;
#23451=ADVANCED_FACE ( 'NONE', ( #39890 ), #54164, .F. ) ;
#23452=CARTESIAN_POINT ( 'NONE',  ( 14.56100101959348692, -277.6553809904083892, -326.6418474436669612 ) ) ;
#23453=CARTESIAN_POINT ( 'NONE',  ( -89.47209198682517695, -279.1258560742897998, -219.1874052828304968 ) ) ;
#23455=CARTESIAN_POINT ( 'NONE',  ( -91.38712892237528251, -299.2815941995733624, -218.5267148475721797 ) ) ;
#23456=CARTESIAN_POINT ( 'NONE',  ( 37.46143141386919950, -285.5971482509502835, -273.8705863856440601 ) ) ;
#23457=CARTESIAN_POINT ( 'NONE',  ( -111.8619470053454137, -292.3541002016450534, -254.3880597077790640 ) ) ;
#23458=CARTESIAN_POINT ( 'NONE',  ( -0.6149505866814742872, -293.4725366883398578, -333.8648693268341958 ) ) ;
#23460=CARTESIAN_POINT ( 'NONE',  ( 10.30210858037631638, -294.0397776248563559, -325.6978596506181702 ) ) ;
#23461=CARTESIAN_POINT ( 'NONE',  ( -111.2404196005671793, -291.3738785194781826, -290.8665263092275381 ) ) ;
#23463=CARTESIAN_POINT ( 'NONE',  ( -67.35571448802896555, -280.2992433411040452, -203.6912722524530466 ) ) ;
#23464=CARTESIAN_POINT ( 'NONE',  ( 30.46245456227480730, -297.8026840890044014, -193.6823012627349101 ) ) ;
#23465=CARTESIAN_POINT ( 'NONE',  ( 39.24666770736248367, -288.2899038058766905, -277.2556592056690192 ) ) ;
#23466=CARTESIAN_POINT ( 'NONE',  ( -38.91548642885345544, -289.4046705166271067, -347.3238848786846802 ) ) ;
#23467=CARTESIAN_POINT ( 'NONE',  ( -81.49473269013293475, -285.7655515821485324, -212.2010182383625931 ) ) ;
#23468=DIRECTION ( 'NONE',  ( 0.000000000000000000, 0.000000000000000000, -1.000000000000000000 ) ) ;
#23469=CARTESIAN_POINT ( 'NONE',  ( 199.9777737730213119, 292.7032345016298791, -82.77980196592716311 ) ) ;
#23470=CARTESIAN_POINT ( 'NONE',  ( 160.4524113272230181, 217.9076703733470879, -202.3092286760552554 ) ) ;
#23471=CARTESIAN_POINT ( 'NONE',  ( -21.62828341911615482, -276.0428233677268963, -341.8673366536299909 ) ) ;
#23472=CARTESIAN_POINT ( 'NONE',  ( -59.30063096982176063, -276.2635352555924442, -340.3041764608137214 ) ) ;
#23473=CARTESIAN_POINT ( 'NONE',  ( -114.3205561439198874, -272.2189246291147811, -270.3568838636807641 ) ) ;
#23474=CARTESIAN_POINT ( 'NONE',  ( 46.79431152631179458, 10.63313198298185114, -329.4643313189536116 ) ) ;
#23475=CARTESIAN_POINT ( 'NONE',  ( -79.96542937547629037, -276.3001900730918692, -333.9584828280872557 ) ) ;
#23476=CARTESIAN_POINT ( 'NONE',  ( -55.80212160902548391, -297.0467995301833071, -344.0712723038736272 ) ) ;
#23478=CARTESIAN_POINT ( 'NONE',  ( 6.708358894044986975, -293.1622806422601002, -212.0723476952181841 ) ) ;
#23479=CARTESIAN_POINT ( 'NONE',  ( -65.49238998103280096, -298.4962842910365453, -198.8081086969549460 ) ) ;
#23480=CARTESIAN_POINT ( 'NONE',  ( -36.19182844920897679, -298.5585315653030989, -193.4225628156010828 ) ) ;
#23481=CARTESIAN_POINT ( 'NONE',  ( -106.7074509629423176, -297.0226299362166742, -247.4545826240741917 ) ) ;
#23484=CARTESIAN_POINT ( 'NONE',  ( -71.87099015364437093, -281.5195575060055830, -203.1377934289358507 ) ) ;
#23485=CARTESIAN_POINT ( 'NONE',  ( 15.70656479875309408, -281.8327126843012138, -326.0873101309804269 ) ) ;
#23486=CARTESIAN_POINT ( 'NONE',  ( -107.4080032043713118, -279.3453949281718565, -292.0934459617955667 ) ) ;
#23487=CARTESIAN_POINT ( 'NONE',  ( -105.2797664069807126, -280.7572521816142626, -236.2086864157508330 ) ) ;
#23488=CARTESIAN_POINT ( 'NONE',  ( -63.53523545373780479, -272.1843679650526155, -201.4663940986789896 ) ) ;
#23491=CARTESIAN_POINT ( 'NONE',  ( 17.96313950408061544, -281.0400251356763874, -222.6934809092687715 ) ) ;
#23492=CARTESIAN_POINT ( 'NONE',  ( 37.12620247485178027, -276.1174930344740233, -251.4219970159843456 ) ) ;
#23493=CARTESIAN_POINT ( 'NONE',  ( 36.22568031408611944, -277.7396327974316819, -284.9501956354350227 ) ) ;
#23494=CARTESIAN_POINT ( 'NONE',  ( -112.7208955753931292, -276.9691810318370244, -282.8744383690524273 ) ) ;
#23497=CARTESIAN_POINT ( 'NONE',  ( -16.57048577135595835, -284.7651116773957938, -342.8511553626584600 ) ) ;
#23498=CARTESIAN_POINT ( 'NONE',  ( -75.05409881503862835, -290.7333507131862689, -207.6092600630848040 ) ) ;
#23499=CARTESIAN_POINT ( 'NONE',  ( -20.99753407276626405, -285.6051818535179905, -195.2200438471334962 ) ) ;
#23500=CARTESIAN_POINT ( 'NONE',  ( -103.9340603573664623, -282.3593196420072218, -302.7810863540076980 ) ) ;
#23501=CARTESIAN_POINT ( 'NONE',  ( -15.97864367260608276, -281.3450961218981661, -340.7812481641582849 ) ) ;
#23502=CARTESIAN_POINT ( 'NONE',  ( 30.12517940097567148, -285.2154656458999966, -238.9042528891214658 ) ) ;
#23503=CARTESIAN_POINT ( 'NONE',  ( 9.518319208454666835, -281.9181137974733815, -213.8035582641167025 ) ) ;
#23504=CARTESIAN_POINT ( 'NONE',  ( 168.2163488282115225, 233.8014272134587941, -193.1015290748493385 ) ) ;
#23505=CARTESIAN_POINT ( 'NONE',  ( 25.26132950738688976, -280.5322397052373162, -313.8271366257532122 ) ) ;
#23506=CARTESIAN_POINT ( 'NONE',  ( 29.11463320946414157, -295.0905173511296766, -235.4850882693889957 ) ) ;
#23507=CARTESIAN_POINT ( 'NONE',  ( -66.50191932104934267, -287.6713123427426808, -201.0811782817712583 ) ) ;
#23509=CARTESIAN_POINT ( 'NONE',  ( -41.99026512915360598, -293.9141387681626156, -194.9442429315811580 ) ) ;
#23510=CARTESIAN_POINT ( 'NONE',  ( 37.64300481556626465, -273.5325373231307822, -268.8463010935575426 ) ) ;
#23511=CARTESIAN_POINT ( 'NONE',  ( 32.71345748152251787, -287.1533847503155812, -301.9274562608538304 ) ) ;
#23512=CARTESIAN_POINT ( 'NONE',  ( 35.10587121427636959, -292.1355343636108159, -284.4248949795370436 ) ) ;
#23514=CARTESIAN_POINT ( 'NONE',  ( -76.63353191152623367, -276.2744616560302120, -332.5289114047803309 ) ) ;
#23515=CARTESIAN_POINT ( 'NONE',  ( -111.6094868382501488, -294.7135145379022561, -268.6817049044715873 ) ) ;
#23516=CARTESIAN_POINT ( 'NONE',  ( -110.7983922557024385, -291.8203126241483005, -273.9496247675755285 ) ) ;
#23519=CARTESIAN_POINT ( 'NONE',  ( 37.08935566046246635, -291.8191707954212006, -253.4880171775016890 ) ) ;
#23520=CARTESIAN_POINT ( 'NONE',  ( 33.85909981965790649, -289.4082111814997802, -289.9645185982417388 ) ) ;
#23521=CARTESIAN_POINT ( 'NONE',  ( -107.8664126688921101, -288.4282312385181513, -298.6496126896894907 ) ) ;
#23522=CARTESIAN_POINT ( 'NONE',  ( 35.85866687328238811, -288.8785630501906780, -262.8059086996532869 ) ) ;
#23524=CARTESIAN_POINT ( 'NONE',  ( 11.23365076474864921, -287.5481937864954602, -215.5844037493591259 ) ) ;
#23525=CARTESIAN_POINT ( 'NONE',  ( -6.448457155595283652, -296.6283075887543532, -339.0925834451596188 ) ) ;
#23527=CARTESIAN_POINT ( 'NONE',  ( -75.45274609958812562, -290.7538245273672715, -336.8107748187499055 ) ) ;
#23528=CARTESIAN_POINT ( 'NONE',  ( -25.62591083777251910, -278.2208301491812676, -195.9222364639070975 ) ) ;
#23529=CARTESIAN_POINT ( 'NONE',  ( -62.39509707870276856, -277.7024976222360237, -343.2052629585372188 ) ) ;
#23530=CARTESIAN_POINT ( 'NONE',  ( -88.91413412554706497, -279.0173557941939180, -213.2119417590596129 ) ) ;
#23531=CARTESIAN_POINT ( 'NONE',  ( -72.46065280030273925, -299.5648933895737400, -204.4792619127440219 ) ) ;
#23532=CARTESIAN_POINT ( 'NONE',  ( -33.10077252724253327, -284.1052760838761628, -195.4299285963734008 ) ) ;
#23534=CARTESIAN_POINT ( 'NONE',  ( -38.34717579188062331, -278.1790047405590940, -196.1201137718282723 ) ) ;
#23535=CARTESIAN_POINT ( 'NONE',  ( -33.19545634619050389, -280.9997982591336836, -345.2592196878421760 ) ) ;
#23537=CARTESIAN_POINT ( 'NONE',  ( -48.41270154851726915, -275.6703622962211853, -345.9138047990541622 ) ) ;
#23539=CARTESIAN_POINT ( 'NONE',  ( -103.3809674688449007, -297.6317489508992935, -303.1799350553461636 ) ) ;
#23540=CARTESIAN_POINT ( 'NONE',  ( -81.39528169475926234, -282.5558487563033623, -333.2013193362076322 ) ) ;
#23541=CARTESIAN_POINT ( 'NONE',  ( -101.4262312441805278, -297.9763214060499195, -234.9128272036355440 ) ) ;
#23542=CARTESIAN_POINT ( 'NONE',  ( -112.4921638422901111, -274.1551650546416568, -256.2574839311059236 ) ) ;
#23543=CARTESIAN_POINT ( 'NONE',  ( -6.271483248217240458, -276.2990689888347333, -336.4561211331753725 ) ) ;
#23544=CARTESIAN_POINT ( 'NONE',  ( 22.94900238363420542, -296.1610629447498582, -314.9708909259636016 ) ) ;
#23545=CARTESIAN_POINT ( 'NONE',  ( 10.22961282020613716, -288.5834803138327516, -330.9762068367739403 ) ) ;
#23546=CARTESIAN_POINT ( 'NONE',  ( -81.37939867735384780, -277.5382371918254307, -208.9608305079144941 ) ) ;
#23547=CARTESIAN_POINT ( 'NONE',  ( -100.6818060166591806, -289.8072537748542459, -314.1450304451814191 ) ) ;
#23549=CARTESIAN_POINT ( 'NONE',  ( -107.1801026994411075, -289.3176068332623458, -292.5744800926738094 ) ) ;
#23550=CARTESIAN_POINT ( 'NONE',  ( 35.81623944262175741, -291.3392100435644920, -253.7832622219589496 ) ) ;
#23553=CARTESIAN_POINT ( 'NONE',  ( -96.80779806890419081, -290.6533868864454462, -227.8282724568342132 ) ) ;
#23555=CARTESIAN_POINT ( 'NONE',  ( -54.92239823472858973, -286.7726919984503979, -195.6366958278105983 ) ) ;
#23556=CARTESIAN_POINT ( 'NONE',  ( -82.08285599513421005, -286.1948066931273615, -326.5171145203363494 ) ) ;
#23557=CARTESIAN_POINT ( 'NONE',  ( 36.14094849259062414, -292.8925313064224838, -292.7474091686557358 ) ) ;
#23559=CARTESIAN_POINT ( 'NONE',  ( 11.19276923560565606, -283.7115161180572613, -329.5710712945125351 ) ) ;
#23560=CARTESIAN_POINT ( 'NONE',  ( -109.4207908131238725, -284.5389947961608641, -258.7232033088644130 ) ) ;
#23561=CARTESIAN_POINT ( 'NONE',  ( 36.09560996715755010, -276.9192415102693303, -274.3226278999974852 ) ) ;
#23562=CARTESIAN_POINT ( 'NONE',  ( -30.63462814121000832, -290.1574822226092465, -196.0182502149615686 ) ) ;
#23563=CARTESIAN_POINT ( 'NONE',  ( 22.61400874048008092, -273.7590846117007004, -228.0020968140500202 ) ) ;
#23565=CARTESIAN_POINT ( 'NONE',  ( -78.59295187722810283, -208.2960365483323244, -357.4574221067172743 ) ) ;
#23566=CARTESIAN_POINT ( 'NONE',  ( -36.27899912000115989, -294.7059279999600676, -347.3457386169311008 ) ) ;
#23567=CARTESIAN_POINT ( 'NONE',  ( -19.49382052750853234, -288.2036628583100537, -198.0924014539831148 ) ) ;
#23568=CARTESIAN_POINT ( 'NONE',  ( -92.46523033144005410, -296.8984075073406075, -323.6798663498537394 ) ) ;
#23569=CARTESIAN_POINT ( 'NONE',  ( -33.24122393159622391, -286.7564215905910032, -197.3243884534402639 ) ) ;
#23570=CARTESIAN_POINT ( 'NONE',  ( -111.8546203887142809, -277.8431189493210809, -251.8506538120986988 ) ) ;
#23571=CARTESIAN_POINT ( 'NONE',  ( 26.40374852036649855, -293.6350272628185962, -227.2578057689176489 ) ) ;
#23572=CARTESIAN_POINT ( 'NONE',  ( -0.2990882997848233193, -284.6788213662377984, -204.2543252490236796 ) ) ;
#23573=CARTESIAN_POINT ( 'NONE',  ( 25.69977724022104226, -294.4699911791835234, -314.5600954182273767 ) ) ;
#23574=CARTESIAN_POINT ( 'NONE',  ( -101.1442168695890160, -291.3721488760276657, -234.7420961536823256 ) ) ;
#23577=CARTESIAN_POINT ( 'NONE',  ( 201.5944599935328370, 289.7950610217533836, -82.37615236527834384 ) ) ;
#23578=CARTESIAN_POINT ( 'NONE',  ( -62.98680599413593484, -287.2442800355714780, -198.4929310210908966 ) ) ;
#23579=CARTESIAN_POINT ( 'NONE',  ( 44.71564893372296723, -273.0523547857346784, -270.3937649182068412 ) ) ;
#23581=CARTESIAN_POINT ( 'NONE',  ( -24.02276734314449769, -281.7983367913138864, -342.4501747263089442 ) ) ;
#23582=CARTESIAN_POINT ( 'NONE',  ( -106.3283173799112262, -277.7784303942466977, -304.6364541672766109 ) ) ;
#23583=CARTESIAN_POINT ( 'NONE',  ( 32.77948886033910014, -283.2105256915716609, -244.0774173914742846 ) ) ;
#23584=CARTESIAN_POINT ( 'NONE',  ( -107.4366190058017452, -267.2042186947507503, -306.5197711127555067 ) ) ;
#23585=CARTESIAN_POINT ( 'NONE',  ( -70.23306157161640328, -282.0517770589909787, -339.3447723352304592 ) ) ;
#23586=CARTESIAN_POINT ( 'NONE',  ( 37.19670806341779468, -285.5095962568583445, -265.5042523385958475 ) ) ;
#23587=CARTESIAN_POINT ( 'NONE',  ( 30.13923431255202701, -276.9616627408163367, -235.9136367270153869 ) ) ;
#23588=CARTESIAN_POINT ( 'NONE',  ( -70.50107694906718336, -298.0950670391416111, -205.2438596243530355 ) ) ;
#23589=CARTESIAN_POINT ( 'NONE',  ( -2.927558067487958215, -293.2720838604775508, -335.2988597454757951 ) ) ;
#23590=CARTESIAN_POINT ( 'NONE',  ( -104.8820951776833112, -278.7271707259505433, -307.1253373111703695 ) ) ;
#23591=CARTESIAN_POINT ( 'NONE',  ( -37.80975951750138364, -277.0581396920400721, -343.3720703023441843 ) ) ;
#23592=CARTESIAN_POINT ( 'NONE',  ( -112.7668337591357215, -273.8096200108537914, -256.2013796315380887 ) ) ;
#23593=CARTESIAN_POINT ( 'NONE',  ( -104.7106323510944037, -276.9963648012179078, -307.0069837805684188 ) ) ;
#23594=CARTESIAN_POINT ( 'NONE',  ( -84.39908107233776491, -219.2962774960793979, -352.3863144506248091 ) ) ;
#23595=CARTESIAN_POINT ( 'NONE',  ( 10.67323324769085247, -274.3889048359586127, -328.0435385926230083 ) ) ;
#23596=CARTESIAN_POINT ( 'NONE',  ( -111.7051398859757683, -298.1988547736701776, -252.7916808038707188 ) ) ;
#23599=CARTESIAN_POINT ( 'NONE',  ( -68.74690798376259693, -285.2194302501843595, -339.5684534487003248 ) ) ;
#23600=CARTESIAN_POINT ( 'NONE',  ( -77.09755191397748320, -284.8527762138687649, -208.9547915133703668 ) ) ;
#23601=CARTESIAN_POINT ( 'NONE',  ( -103.8608281804737743, -276.5228849773250204, -302.4426294836409852 ) ) ;
#23602=CARTESIAN_POINT ( 'NONE',  ( -74.39308335077448930, -285.4104486083722918, -334.7474456918561714 ) ) ;
#23603=CARTESIAN_POINT ( 'NONE',  ( -106.1548236246012351, -277.3826046744385394, -243.8466796971943609 ) ) ;
#23604=CARTESIAN_POINT ( 'NONE',  ( -1.306342928227328892, -277.6422220336684745, -334.2596121709232762 ) ) ;
#23606=CARTESIAN_POINT ( 'NONE',  ( -34.04417049204357681, -274.5870931576932890, -197.3740318639470956 ) ) ;
#23607=TOROIDAL_SURFACE ( 'NONE', #6989, 5.654241149514406040, 0.5000000000000000000 ) ;
#23608=CARTESIAN_POINT ( 'NONE',  ( 33.02097094963124846, -281.9604002381283294, -239.4863169495665431 ) ) ;
#23609=CARTESIAN_POINT ( 'NONE',  ( 38.73291562117786668, -281.8962747702636875, -258.5188183353056957 ) ) ;
#23611=ORIENTED_EDGE ( 'NONE', *, *, #88201, .T. ) ;
#23613=CARTESIAN_POINT ( 'NONE',  ( 9.035670697446112953, -288.5415056901899788, -210.4491412741920158 ) ) ;
#23614=CARTESIAN_POINT ( 'NONE',  ( -95.41100991186628733, -296.3742644784641129, -225.8372593236062755 ) ) ;
#23615=CARTESIAN_POINT ( 'NONE',  ( -36.37131084586341956, -291.4126097395954957, -193.4561581629470766 ) ) ;
#23616=CARTESIAN_POINT ( 'NONE',  ( 23.30962994678129974, -286.6097956958180362, -312.2417321816748768 ) ) ;
#23617=CARTESIAN_POINT ( 'NONE',  ( -29.12520881523634486, -287.5207084020196362, -343.4902106005949918 ) ) ;
#23618=CARTESIAN_POINT ( 'NONE',  ( -79.55010188561553264, -286.6731226058781772, -210.2522209410640812 ) ) ;
#23619=CARTESIAN_POINT ( 'NONE',  ( -73.16458745200385749, -275.5268462611056179, -336.2674725587354487 ) ) ;
#23620=CARTESIAN_POINT ( 'NONE',  ( -43.14193866221108209, -287.5241126698760468, -346.3400469592653508 ) ) ;
#23621=CARTESIAN_POINT ( 'NONE',  ( -62.55372808273050822, -287.7242411624579290, -199.7257564820693005 ) ) ;
#23622=CARTESIAN_POINT ( 'NONE',  ( -74.77335587903566250, -287.5491056496915121, -335.5447016130929114 ) ) ;
#23623=CARTESIAN_POINT ( 'NONE',  ( 10.07011855260182465, -283.3212931710614271, -326.2447316867698532 ) ) ;
#23624=CARTESIAN_POINT ( 'NONE',  ( -96.91134893754593804, -293.1791205058588616, -224.4983202420237660 ) ) ;
#23626=CARTESIAN_POINT ( 'NONE',  ( 144.2857639756989272, -299.5541904835127980, -189.7068768330456123 ) ) ;
#23627=CARTESIAN_POINT ( 'NONE',  ( -112.8982735732997185, -298.4814843182186905, -269.6411149513203895 ) ) ;
#23628=EDGE_CURVE ( 'NONE', #30942, #49115, #66326, .T. ) ;
#23629=CARTESIAN_POINT ( 'NONE',  ( 20.65017696660128266, -280.1227418842138377, -225.7364488081120157 ) ) ;
#23630=CARTESIAN_POINT ( 'NONE',  ( 12.65758128666331039, -278.7492407457295371, -214.4587700520113458 ) ) ;
#23631=CARTESIAN_POINT ( 'NONE',  ( 1.678608228784536971, -293.7413621927649956, -336.5545795642934195 ) ) ;
#23632=CARTESIAN_POINT ( 'NONE',  ( -41.89759333070529124, -296.3936530147983603, -196.7018738034329886 ) ) ;
#23633=CARTESIAN_POINT ( 'NONE',  ( 18.49956782502580666, -274.3215419306684453, -319.6049986156690466 ) ) ;
#23634=CARTESIAN_POINT ( 'NONE',  ( -92.55013752300727958, -297.1794518962731217, -318.8716520887538195 ) ) ;
#23636=CARTESIAN_POINT ( 'NONE',  ( -3.770512523477011602, -296.9451216367822894, -194.0629393281858768 ) ) ;
#23637=CARTESIAN_POINT ( 'NONE',  ( -100.7946061276290521, -294.2339211616690591, -312.2618534305539697 ) ) ;
#23638=CARTESIAN_POINT ( 'NONE',  ( 21.45372518083881630, -294.3609187266864637, -226.1064811485536836 ) ) ;
#23640=CARTESIAN_POINT ( 'NONE',  ( 30.97553211781579208, -294.0061167409050995, -244.1817844366976544 ) ) ;
#23642=CARTESIAN_POINT ( 'NONE',  ( -107.4879428154368242, -282.9304951549263478, -242.6891434258418485 ) ) ;
#23643=CARTESIAN_POINT ( 'NONE',  ( 3.816386721421738848, -294.4806905750288024, -330.6521777417710837 ) ) ;
#23644=CARTESIAN_POINT ( 'NONE',  ( -98.04442191513393823, -283.9191831028469437, -317.7338904119175709 ) ) ;
#23645=CARTESIAN_POINT ( 'NONE',  ( -36.78813083755425595, -281.9792085351709261, -194.7903407221597547 ) ) ;
#23646=CARTESIAN_POINT ( 'NONE',  ( 0.2771659567876044727, -286.2057095461482277, -203.1853325412872664 ) ) ;
#23647=CARTESIAN_POINT ( 'NONE',  ( -103.2700900060842457, -288.0797640030843354, -305.8755136904109122 ) ) ;
#23648=CARTESIAN_POINT ( 'NONE',  ( -54.49178911615187815, -280.7666405000204009, -345.3538533559490702 ) ) ;
#23649=CARTESIAN_POINT ( 'NONE',  ( 19.05086839509208829, -285.5723561561008523, -223.2127284513679228 ) ) ;
#23650=CARTESIAN_POINT ( 'NONE',  ( -109.1794400119410966, -289.8151225119756873, -243.3615450881882794 ) ) ;
#23652=CARTESIAN_POINT ( 'NONE',  ( -6.411260363033599141, -296.2390725767519939, -337.3667021773065926 ) ) ;
#23653=CARTESIAN_POINT ( 'NONE',  ( -111.5183373542898124, -280.2092604009340562, -251.9652789025995787 ) ) ;
#23654=CARTESIAN_POINT ( 'NONE',  ( -1.510962052055676796, -292.5997228194920012, -336.6671985461200052 ) ) ;
#23655=CARTESIAN_POINT ( 'NONE',  ( 31.09160564204640309, -280.8774598790478194, -244.7411384554898746 ) ) ;
#23656=CARTESIAN_POINT ( 'NONE',  ( -37.68684804680010814, -295.2230053076495437, -347.3734229007654335 ) ) ;
#23657=CARTESIAN_POINT ( 'NONE',  ( -94.70697914160658115, -283.3089630194299389, -221.1040267450195245 ) ) ;
#23658=CARTESIAN_POINT ( 'NONE',  ( -91.64376406224226912, -281.2790824145236570, -218.5540490039744270 ) ) ;
#23660=CARTESIAN_POINT ( 'NONE',  ( -5.449845175431134336, -293.6807130319604084, -336.3015827400045623 ) ) ;
#23661=CARTESIAN_POINT ( 'NONE',  ( -94.61386983468875655, -271.2244966725415338, -221.6594127210166505 ) ) ;
#23664=CARTESIAN_POINT ( 'NONE',  ( 36.77603671812038044, -283.6517312517378286, -279.6381901162179702 ) ) ;
#23665=CARTESIAN_POINT ( 'NONE',  ( -100.2226289584829857, -295.5478707892269767, -307.6625933678001843 ) ) ;
#23667=CARTESIAN_POINT ( 'NONE',  ( -4.829096099716524648, -274.1237833571632905, -337.9475929042657754 ) ) ;
#23668=CARTESIAN_POINT ( 'NONE',  ( -18.57948399627296965, -273.4848991087040986, -195.7935311083072349 ) ) ;
#23669=CARTESIAN_POINT ( 'NONE',  ( -31.84537720400900440, -290.2994674338366394, -346.7225023559164470 ) ) ;
#23670=CARTESIAN_POINT ( 'NONE',  ( -108.3509113692800270, -290.1620906597057115, -287.2930972950791215 ) ) ;
#23671=CARTESIAN_POINT ( 'NONE',  ( -22.06944292388590156, -281.7713492211050834, -198.2153180721255694 ) ) ;
#23672=CARTESIAN_POINT ( 'NONE',  ( -43.56973256083086454, -275.5724403804326812, -196.7731117260306917 ) ) ;
#23673=CARTESIAN_POINT ( 'NONE',  ( -36.99111024483472221, -278.8515612959367900, -196.9648810698413968 ) ) ;
#23674=CARTESIAN_POINT ( 'NONE',  ( -21.19836542798471157, -278.8453654253348191, -343.6565583733109861 ) ) ;
#23676=CARTESIAN_POINT ( 'NONE',  ( -85.80658563474980838, -273.2352961210023636, -210.5267225455737332 ) ) ;
#23677=CARTESIAN_POINT ( 'NONE',  ( -58.07909303802962597, -293.7024421546607300, -198.8140131671668485 ) ) ;
#23681=CARTESIAN_POINT ( 'NONE',  ( 21.26903376294168524, -291.0365544468612029, -222.3497926835745488 ) ) ;
#23682=CARTESIAN_POINT ( 'NONE',  ( -105.4713553622504776, -272.4137758091697492, -243.8333662622118823 ) ) ;
#23685=CARTESIAN_POINT ( 'NONE',  ( 14.94882903990264822, -294.2932183090470630, -214.7151357154085076 ) ) ;
#23686=CARTESIAN_POINT ( 'NONE',  ( -55.63300648810263738, -300.3376638359844719, -190.3683826091709363 ) ) ;
#23687=CARTESIAN_POINT ( 'NONE',  ( 17.29604931729026873, -288.8344578617546858, -219.2076403802323625 ) ) ;
#23688=CARTESIAN_POINT ( 'NONE',  ( 28.36459331370843984, -274.0301895428460170, -306.2843399587681574 ) ) ;
#23689=CARTESIAN_POINT ( 'NONE',  ( 12.49275071668670023, -276.6726242751695395, -214.9939777256952880 ) ) ;
#23690=CARTESIAN_POINT ( 'NONE',  ( -73.30154083974619539, -289.6516149867449599, -205.1249540572253238 ) ) ;
#23691=CARTESIAN_POINT ( 'NONE',  ( -47.96933495990111140, -281.7789060834294332, -195.2924112356211310 ) ) ;
#23693=CARTESIAN_POINT ( 'NONE',  ( -29.44187087593311603, -282.2981713747406616, -343.0855205921752713 ) ) ;
#23694=CARTESIAN_POINT ( 'NONE',  ( -112.9919834803592238, -279.4737202304755783, -282.9518740670446277 ) ) ;
#23695=CARTESIAN_POINT ( 'NONE',  ( -8.204209013251229976, -281.4740211295047629, -341.2623691472579139 ) ) ;
#23696=CARTESIAN_POINT ( 'NONE',  ( -72.72154477837992204, -278.4502987993755596, -338.5012982650375193 ) ) ;
#23697=CARTESIAN_POINT ( 'NONE',  ( -8.131969979251900682, -278.1966032418925465, -340.8699522798682437 ) ) ;
#23698=CARTESIAN_POINT ( 'NONE',  ( -82.08285599513421005, -286.1948066931273615, -326.5171145203363494 ) ) ;
#23701=CARTESIAN_POINT ( 'NONE',  ( -105.5477509207837414, -298.9631972017145927, -239.0441111789417903 ) ) ;
#23702=CARTESIAN_POINT ( 'NONE',  ( -84.87504876384126362, -290.8052159675451662, -326.2385652259831659 ) ) ;
#23703=CARTESIAN_POINT ( 'NONE',  ( -90.26948662756966257, -275.8249925059587326, -323.0700456038410380 ) ) ;
#23704=CARTESIAN_POINT ( 'NONE',  ( -59.70734677668481538, -291.0981220780837475, -342.9817201686347516 ) ) ;
#23705=CARTESIAN_POINT ( 'NONE',  ( -33.49478737170256437, -291.4504024451915711, -197.3479650668444094 ) ) ;
#23706=CARTESIAN_POINT ( 'NONE',  ( 36.72346799070689372, -287.3215950561159957, -291.2391520109006819 ) ) ;
#23708=CARTESIAN_POINT ( 'NONE',  ( -91.34056130169399523, -282.2365002186331253, -320.6658236015437069 ) ) ;
#23709=CARTESIAN_POINT ( 'NONE',  ( -76.50052936066884968, -291.4424939987589482, -333.4281582862054734 ) ) ;
#23710=CARTESIAN_POINT ( 'NONE',  ( -75.05849261621393964, -284.0196463547703729, -207.0511557583419631 ) ) ;
#23711=CARTESIAN_POINT ( 'NONE',  ( -5.358919178937607164, -281.7972513551345628, -204.1920526839323315 ) ) ;
#23712=CARTESIAN_POINT ( 'NONE',  ( 27.25331354631952863, -289.0402782859607669, -311.9357054173046322 ) ) ;
#23713=CARTESIAN_POINT ( 'NONE',  ( -99.22388079738097133, -278.5074608347254070, -309.2961039327813069 ) ) ;
#23714=CARTESIAN_POINT ( 'NONE',  ( 23.66834049785471805, -291.7263794272370205, -224.0169230836491465 ) ) ;
#23715=CARTESIAN_POINT ( 'NONE',  ( -36.57732853976609277, -286.8643449668857670, -193.5133842317157473 ) ) ;
#23716=CARTESIAN_POINT ( 'NONE',  ( 37.96198084474539769, -287.8462400112704245, -254.5213404396648968 ) ) ;
#23717=CARTESIAN_POINT ( 'NONE',  ( -95.92047378970561056, -284.1078156761905120, -313.9217341492939113 ) ) ;
#23720=CARTESIAN_POINT ( 'NONE',  ( 34.27711181027408571, -295.0940647306704250, -245.4830056167927523 ) ) ;
#23721=CARTESIAN_POINT ( 'NONE',  ( 39.21813982612355431, -292.2365499623663823, -270.3270031064367345 ) ) ;
#23722=CARTESIAN_POINT ( 'NONE',  ( 3.254608541759664408, -275.5504116477532079, -331.3147739031238075 ) ) ;
#23723=CARTESIAN_POINT ( 'NONE',  ( -99.83386833973021623, -296.4953568145294867, -225.5499397012155214 ) ) ;
#23724=CARTESIAN_POINT ( 'NONE',  ( 30.11703625713074572, -292.4273791275849135, -300.0263608761631531 ) ) ;
#23725=CARTESIAN_POINT ( 'NONE',  ( -95.23005910177541011, -295.4344117431912196, -224.2426627599575966 ) ) ;
#23726=CARTESIAN_POINT ( 'NONE',  ( -91.97895070757937219, -292.4549808932696351, -221.3331180906272380 ) ) ;
#23727=CARTESIAN_POINT ( 'NONE',  ( 23.19599393104245166, -295.2057403767670962, -311.7949675016975561 ) ) ;
#23729=CARTESIAN_POINT ( 'NONE',  ( -61.03834599168131092, -293.3587371776023360, -341.7492416118952292 ) ) ;
#23730=CARTESIAN_POINT ( 'NONE',  ( -111.4051325982030676, -298.3995686644375951, -282.2571981095354090 ) ) ;
#23731=CARTESIAN_POINT ( 'NONE',  ( -0.8638712076543580975, -289.4966536073875432, -333.9236406160345609 ) ) ;
#23732=CARTESIAN_POINT ( 'NONE',  ( 32.66575191105214060, -277.8950840933381983, -298.3831569637608254 ) ) ;
#23733=CARTESIAN_POINT ( 'NONE',  ( -96.42582866246149820, -277.8943071983611048, -221.7365944833149740 ) ) ;
#23734=CARTESIAN_POINT ( 'NONE',  ( -5.149371496979327389, -273.8134592347573175, -200.5258348918962952 ) ) ;
#23735=CARTESIAN_POINT ( 'NONE',  ( 37.12854104167171698, -279.6088583577912914, -268.5729121899955203 ) ) ;
#23736=CARTESIAN_POINT ( 'NONE',  ( 0.6305054117470390018, -274.9550107430797539, -336.4857164793249922 ) ) ;
#23738=CARTESIAN_POINT ( 'NONE',  ( -94.33554197619169202, -294.5844211212437358, -316.7807452265661823 ) ) ;
#23740=CARTESIAN_POINT ( 'NONE',  ( -6.493500732843245693, -275.1197641780397021, -204.0868298866615760 ) ) ;
#23742=CARTESIAN_POINT ( 'NONE',  ( -100.9272138103576282, -288.0295444183770428, -310.8958990310553645 ) ) ;
#23743=CARTESIAN_POINT ( 'NONE',  ( -112.8679962522325866, -290.3638129636675558, -285.4205680058415169 ) ) ;
#23744=CARTESIAN_POINT ( 'NONE',  ( 6.761243456491912163, -300.5815312243726680, -194.9911137133431964 ) ) ;
#23745=CARTESIAN_POINT ( 'NONE',  ( -110.9499677108039037, -294.3775424395805089, -283.9174618738385334 ) ) ;
#23746=CARTESIAN_POINT ( 'NONE',  ( 6.823820858814699797, -281.6655426567394329, -333.3035610497407788 ) ) ;
#23748=CARTESIAN_POINT ( 'NONE',  ( 26.02162632492521155, -280.0928590006643617, -310.5826702957890575 ) ) ;
#23750=CARTESIAN_POINT ( 'NONE',  ( -62.92483046979299388, -290.5063902385302299, -201.5669761773716573 ) ) ;
#23751=CARTESIAN_POINT ( 'NONE',  ( -92.60007452029728370, -281.9939301119690640, -319.9521959839975125 ) ) ;
#23754=CARTESIAN_POINT ( 'NONE',  ( 36.69218430280204757, -291.3968879084102923, -258.2812851779880816 ) ) ;
#23755=CARTESIAN_POINT ( 'NONE',  ( -32.34627376723635450, -278.5883910844883076, -344.0423731885952634 ) ) ;
#23756=CARTESIAN_POINT ( 'NONE',  ( -65.09395149291948712, -284.6118741767489269, -341.7742756927728465 ) ) ;
#23757=CARTESIAN_POINT ( 'NONE',  ( -5.694686395241257415, -272.5449236736599801, -201.7478486865377079 ) ) ;
#23758=CARTESIAN_POINT ( 'NONE',  ( 33.08553933276996872, -277.2582394440208304, -291.7444443146456479 ) ) ;
#23759=CARTESIAN_POINT ( 'NONE',  ( 25.51952530406399688, -276.8684533413307918, -307.7919617326492698 ) ) ;
#23760=CARTESIAN_POINT ( 'NONE',  ( -106.1029658601182604, -286.9457713872822069, -240.2830571392789523 ) ) ;
#23763=CARTESIAN_POINT ( 'NONE',  ( -111.0908949349528712, -270.9825380859393249, -270.3411330354564370 ) ) ;
#23764=CARTESIAN_POINT ( 'NONE',  ( -53.29131893547408083, -295.0844389604874323, -345.7456665325554468 ) ) ;
#23765=CARTESIAN_POINT ( 'NONE',  ( -24.89175949740537064, -288.1914903908325982, -196.7094422370003315 ) ) ;
#23767=CARTESIAN_POINT ( 'NONE',  ( -111.2869819898779866, -293.6237833571632905, -305.9350535429201159 ) ) ;
#23768=CARTESIAN_POINT ( 'NONE',  ( -101.6245809791751640, -278.0250773646622520, -228.4415664899898388 ) ) ;
#23769=CARTESIAN_POINT ( 'NONE',  ( 8.387283476604746824, -291.0659102710815773, -209.3419860969198396 ) ) ;
#23770=CARTESIAN_POINT ( 'NONE',  ( -107.1956738927552095, -286.3830719421417825, -246.7250458566439875 ) ) ;
#23771=CARTESIAN_POINT ( 'NONE',  ( -52.05036797764275036, -281.6216019020221211, -197.7715789073788528 ) ) ;
#23772=CARTESIAN_POINT ( 'NONE',  ( -10.22021151092482683, -287.8244532225228909, -198.8692541545776464 ) ) ;
#23773=CARTESIAN_POINT ( 'NONE',  ( -34.75266722667074504, -285.0198105566751678, -345.3291987317878124 ) ) ;
#23774=CARTESIAN_POINT ( 'NONE',  ( 31.85621553845096443, -276.1538370432323859, -304.2560587003409296 ) ) ;
#23775=CARTESIAN_POINT ( 'NONE',  ( -85.10845996581620909, -295.4095287780866101, -212.9335309116574138 ) ) ;
#23776=CARTESIAN_POINT ( 'NONE',  ( -100.2477601903501920, -278.9730484463010498, -225.9558523943842658 ) ) ;
#23777=CARTESIAN_POINT ( 'NONE',  ( -111.2307951829731678, -298.3500433393001003, -279.8124643945582193 ) ) ;
#23780=CARTESIAN_POINT ( 'NONE',  ( -85.33152481854864391, -275.9090924074130839, -210.2361428286349110 ) ) ;
#23781=CARTESIAN_POINT ( 'NONE',  ( -26.40771704191215008, -296.3272358670997733, -194.5997318284844084 ) ) ;
#23783=CARTESIAN_POINT ( 'NONE',  ( -110.4125176284502885, -278.0922414299042202, -267.8999406243838166 ) ) ;
#23784=CARTESIAN_POINT ( 'NONE',  ( -13.20223463151127063, -275.5639970889189385, -197.6610841212505534 ) ) ;
#23785=CARTESIAN_POINT ( 'NONE',  ( 22.33276463728777728, -281.2606203925236628, -318.6703453541426825 ) ) ;
#23786=CARTESIAN_POINT ( 'NONE',  ( -12.93283279051736301, -290.4906883977004668, -340.2337249750351020 ) ) ;
#23787=CARTESIAN_POINT ( 'NONE',  ( -34.80774276975866854, -299.6034472235986641, -194.0538049768059921 ) ) ;
#23788=CARTESIAN_POINT ( 'NONE',  ( -95.28089541048503008, -298.4382944112228415, -220.1714697068004511 ) ) ;
#23789=CARTESIAN_POINT ( 'NONE',  ( -69.83615561411666306, -293.6234967448971815, -202.9367386652224070 ) ) ;
#23790=CARTESIAN_POINT ( 'NONE',  ( 36.50880623550769855, -279.7075511326453352, -282.4495892469234377 ) ) ;
#23791=CARTESIAN_POINT ( 'NONE',  ( -4.953634996015651382, -282.4021334475221465, -203.3362909475473828 ) ) ;
#23792=CARTESIAN_POINT ( 'NONE',  ( -93.82132065097373186, -295.3091709421734095, -221.8506269889319640 ) ) ;
#23793=CARTESIAN_POINT ( 'NONE',  ( -95.22238364596634597, -286.8286742636647659, -220.7212164923518856 ) ) ;
#23794=CARTESIAN_POINT ( 'NONE',  ( -74.88597072180587588, -288.4850991617178124, -333.3413654865399280 ) ) ;
#23795=CARTESIAN_POINT ( 'NONE',  ( -98.37663915457927999, -248.8749983746587588, -334.1288200131682515 ) ) ;
#23797=CARTESIAN_POINT ( 'NONE',  ( -59.87099359773471008, -287.9132215709267939, -343.3750702615831756 ) ) ;
#23798=CARTESIAN_POINT ( 'NONE',  ( 26.38790659474636868, -286.7301904746042283, -234.6118299107389475 ) ) ;
#23800=CARTESIAN_POINT ( 'NONE',  ( -83.68542741185271439, -284.7507385847470118, -331.5322490186136406 ) ) ;
#23801=CARTESIAN_POINT ( 'NONE',  ( 29.17527318117884150, -276.2913504179543338, -300.4871822534802845 ) ) ;
#23803=CARTESIAN_POINT ( 'NONE',  ( -76.99760560997145831, -290.4547072366088400, -204.6576534808791621 ) ) ;
#23804=CARTESIAN_POINT ( 'NONE',  ( -10.72951485012345074, -283.3655723005207392, -342.5641011175051176 ) ) ;
#23805=CARTESIAN_POINT ( 'NONE',  ( 36.52555394281589685, -283.3139965145331303, -289.5010377970299942 ) ) ;
#23806=CARTESIAN_POINT ( 'NONE',  ( -31.63362043503224186, -283.3152623811682247, -347.1413160497097010 ) ) ;
#23807=CARTESIAN_POINT ( 'NONE',  ( 0.3999504757506849861, -280.5698389978297769, -207.8160622513621547 ) ) ;
#23808=CARTESIAN_POINT ( 'NONE',  ( -53.28691492658257545, -295.3380690714490129, -200.3538533559491555 ) ) ;
#23809=CARTESIAN_POINT ( 'NONE',  ( -112.0640318895732719, -271.7261958592908400, -296.4135090774117316 ) ) ;
#23811=CARTESIAN_POINT ( 'NONE',  ( 35.61557228249901641, -277.3373698464109793, -253.6526428978296792 ) ) ;
#23812=CARTESIAN_POINT ( 'NONE',  ( 179.1553158749216266, 254.2886184646079357, -166.4193513437393790 ) ) ;
#23813=CARTESIAN_POINT ( 'NONE',  ( -41.86637595129381140, -297.3422149966701227, -197.3993473282040725 ) ) ;
#23814=CARTESIAN_POINT ( 'NONE',  ( 15.40054671173733247, -292.2810732461673524, -214.2720501491700702 ) ) ;
#23815=CARTESIAN_POINT ( 'NONE',  ( 201.7602898703672736, 289.7935802246685171, -82.39453363523685425 ) ) ;
#23816=CARTESIAN_POINT ( 'NONE',  ( -35.82431374170981542, -296.6455330352716828, -193.9507017958873973 ) ) ;
#23817=CARTESIAN_POINT ( 'NONE',  ( -23.65659818303267059, -287.2743562672910116, -342.9334358167427013 ) ) ;
#23818=CARTESIAN_POINT ( 'NONE',  ( -71.47805722691788333, -297.3683545409638214, -336.2963095267152767 ) ) ;
#23819=CARTESIAN_POINT ( 'NONE',  ( -73.81482698521389807, -286.8722041519692425, -206.5424903439755724 ) ) ;
#23821=CARTESIAN_POINT ( 'NONE',  ( -94.46843459369449647, -296.7953301135331117, -321.6579492710721979 ) ) ;
#23822=CARTESIAN_POINT ( 'NONE',  ( -101.0480484625467597, -285.5347574658555914, -234.4874666514279227 ) ) ;
#23823=CARTESIAN_POINT ( 'NONE',  ( -14.93901213210802581, -297.1216951677442921, -193.7626547343421919 ) ) ;
#23824=CARTESIAN_POINT ( 'NONE',  ( -53.36564568420788390, -292.6546361128370108, -195.1576014967284038 ) ) ;
#23825=CARTESIAN_POINT ( 'NONE',  ( 20.32840346640906759, -293.3541058025260782, -219.4129714714107422 ) ) ;
#23826=CARTESIAN_POINT ( 'NONE',  ( -94.10294619750740708, -290.0695529661919636, -316.2649407992306010 ) ) ;
#23829=CARTESIAN_POINT ( 'NONE',  ( 51.75226373859299400, -301.0166613338370780, -194.5684141701167107 ) ) ;
#23830=CARTESIAN_POINT ( 'NONE',  ( 36.85032307720787514, -274.5869354967246636, -289.4281684230728047 ) ) ;
#23832=CARTESIAN_POINT ( 'NONE',  ( 26.01264011972551415, -275.6376536612108907, -314.1082674476651846 ) ) ;
#23833=CARTESIAN_POINT ( 'NONE',  ( -41.89199681228512873, -296.4736465157424732, -196.8083984324122753 ) ) ;
#23834=CARTESIAN_POINT ( 'NONE',  ( -108.8138658240379186, -280.6739260031801564, -250.2491787424162055 ) ) ;
#23835=CARTESIAN_POINT ( 'NONE',  ( 14.57858332972057092, -274.4520077790725168, -323.4906689658292862 ) ) ;
#23836=CARTESIAN_POINT ( 'NONE',  ( -109.6697496110946730, -297.9209907192684454, -257.8797813783895663 ) ) ;
#23837=CARTESIAN_POINT ( 'NONE',  ( -34.04203350448968735, -275.0359254128838415, -197.2001950198926181 ) ) ;
#23838=CARTESIAN_POINT ( 'NONE',  ( -112.8581325102493338, -274.4192598553474340, -261.9205935356417854 ) ) ;
#23839=CARTESIAN_POINT ( 'NONE',  ( -5.779709832144479087, -272.4851952159589246, -201.9341673327492970 ) ) ;
#23840=CARTESIAN_POINT ( 'NONE',  ( 16.23949007678421808, -294.9173058159784091, -320.0898694699145608 ) ) ;
#23841=CARTESIAN_POINT ( 'NONE',  ( -72.89583931315375764, -290.1464168377394230, -205.8734492928335840 ) ) ;
#23843=CARTESIAN_POINT ( 'NONE',  ( -91.28141809152558039, -278.2864630770181975, -325.2994934917702494 ) ) ;
#23844=CARTESIAN_POINT ( 'NONE',  ( 35.10635481474194819, -275.8423480909079331, -279.7242288040310427 ) ) ;
#23846=CARTESIAN_POINT ( 'NONE',  ( -64.35728263601791355, -284.3916973768498906, -198.7687176775378362 ) ) ;
#23847=CARTESIAN_POINT ( 'NONE',  ( -47.36136915731026420, -297.1793749862714549, -344.8569880512051213 ) ) ;
#23849=CARTESIAN_POINT ( 'NONE',  ( -83.74240713423068883, -284.5937038152087553, -213.7305055269242757 ) ) ;
#23850=CARTESIAN_POINT ( 'NONE',  ( -24.86361577729069339, -280.8933118845253034, -344.5376624190648727 ) ) ;
#23851=CARTESIAN_POINT ( 'NONE',  ( -46.04925959493782983, -275.4037982373302498, -343.9117833643645099 ) ) ;
#23852=CARTESIAN_POINT ( 'NONE',  ( 35.60698321438832181, -274.0000920151603623, -260.6727478587579299 ) ) ;
#23853=CARTESIAN_POINT ( 'NONE',  ( -7.896232487481309903, -282.4379590160257862, -201.3285514889731758 ) ) ;
#23854=CARTESIAN_POINT ( 'NONE',  ( 32.48062166773370052, -277.0557994643210122, -292.9879578831901767 ) ) ;
#23855=DIRECTION ( 'NONE',  ( -1.000000000000000000, -0.000000000000000000, -0.000000000000000000 ) ) ;
#23856=CARTESIAN_POINT ( 'NONE',  ( -13.29542512518735364, -272.7592449605619436, -198.0547069756708822 ) ) ;
#23857=CARTESIAN_POINT ( 'NONE',  ( 11.77451335985401748, -282.7326330422181968, -213.4609774177922645 ) ) ;
#23859=CARTESIAN_POINT ( 'NONE',  ( -13.18761188330635825, -288.2836691543280381, -198.7657674517327280 ) ) ;
#23861=CARTESIAN_POINT ( 'NONE',  ( -112.3706766292436896, -288.5754777742207580, -268.5316172249676470 ) ) ;
#23863=CARTESIAN_POINT ( 'NONE',  ( -110.2005776581172967, -295.2253174345212869, -279.6409053897473314 ) ) ;
#23864=CARTESIAN_POINT ( 'NONE',  ( -106.2686032546539394, -288.3273018208026315, -298.0663386365166616 ) ) ;
#23865=CARTESIAN_POINT ( 'NONE',  ( 85.37101130053461873, 80.99577858023421584, -298.5812782549759845 ) ) ;
#23867=CARTESIAN_POINT ( 'NONE',  ( 30.81131567701246610, -285.5864111041672686, -236.0409462525921924 ) ) ;
#23868=CARTESIAN_POINT ( 'NONE',  ( 8.304588364289221758, -284.0160764638553132, -328.4165410077273464 ) ) ;
#23869=CARTESIAN_POINT ( 'NONE',  ( -103.5453083600116742, -282.3003944884046632, -307.7646101432980572 ) ) ;
#23870=CARTESIAN_POINT ( 'NONE',  ( -79.53070514208576469, -291.4646717474291222, -210.7249372514021388 ) ) ;
#23871=CARTESIAN_POINT ( 'NONE',  ( 27.38184324191901098, -283.4513769997220720, -305.3787970786149231 ) ) ;
#23872=CARTESIAN_POINT ( 'NONE',  ( 5.695310469968751121, -283.2547879006495464, -329.5254437648013663 ) ) ;
#23873=CARTESIAN_POINT ( 'NONE',  ( -6.280930527751023895, -290.6260054003775508, -339.0170383244702066 ) ) ;
#23874=CARTESIAN_POINT ( 'NONE',  ( -36.18651701771133133, -298.2329201614146541, -193.3610862879390311 ) ) ;
#23875=CARTESIAN_POINT ( 'NONE',  ( -31.95432840838165234, -287.0646614741164626, -345.7803928787717496 ) ) ;
#23876=CARTESIAN_POINT ( 'NONE',  ( 39.38050151352002359, -275.6338790170673860, -276.8959305480021840 ) ) ;
#23877=CARTESIAN_POINT ( 'NONE',  ( -27.92325412946086161, -294.1520733013399536, -196.2610019592440835 ) ) ;
#23879=CARTESIAN_POINT ( 'NONE',  ( -85.28047601435908120, -286.1948066931273615, -330.5268031993605859 ) ) ;
#23880=CARTESIAN_POINT ( 'NONE',  ( -45.47712670929725221, -275.1547142858140091, -345.1380317294898532 ) ) ;
#23882=CARTESIAN_POINT ( 'NONE',  ( -101.6304058046137442, -295.4938606898023750, -229.4538724497002988 ) ) ;
#23883=CARTESIAN_POINT ( 'NONE',  ( -66.90303124352954001, -293.2582770051119496, -202.7403510586119069 ) ) ;
#23884=CARTESIAN_POINT ( 'NONE',  ( 15.52623723758388863, -274.1728276660218739, -219.8014603362215666 ) ) ;
#23885=CARTESIAN_POINT ( 'NONE',  ( -110.3067230472953781, -291.9360447949975992, -280.7865290769095736 ) ) ;
#23886=CARTESIAN_POINT ( 'NONE',  ( -28.08846191411517879, -293.1136004314858496, -197.6618340841534121 ) ) ;
#23887=CARTESIAN_POINT ( 'NONE',  ( -104.4131198845685446, -286.7305219381780717, -238.9442005070774542 ) ) ;
#23888=CARTESIAN_POINT ( 'NONE',  ( -11.37072441228891861, -293.8091242230677267, -198.4437398750833665 ) ) ;
#23889=CARTESIAN_POINT ( 'NONE',  ( 6.201724264528955644, -293.9450042304076760, -207.4542943158702997 ) ) ;
#23890=CARTESIAN_POINT ( 'NONE',  ( -7.990256111431073727, -294.4899406038641700, -337.2140004973140321 ) ) ;
#23891=CARTESIAN_POINT ( 'NONE',  ( 2.392167251682307594, -290.5198157390677807, -333.9710262581976394 ) ) ;
#23892=CARTESIAN_POINT ( 'NONE',  ( 24.25637975933156198, -282.3337561422110298, -316.5636780708224478 ) ) ;
#23893=CARTESIAN_POINT ( 'NONE',  ( -84.30199401848265950, -295.4915915241630842, -211.1661435939996920 ) ) ;
#23894=CARTESIAN_POINT ( 'NONE',  ( -67.18710026026457172, -285.5048218637452351, -199.3804720608231946 ) ) ;
#23895=CARTESIAN_POINT ( 'NONE',  ( 10.74240339485621476, -278.3634436810751822, -327.4554766186412280 ) ) ;
#23896=CARTESIAN_POINT ( 'NONE',  ( -62.68565492269070916, -284.5098659060736850, -201.4243077839427656 ) ) ;
#23897=CARTESIAN_POINT ( 'NONE',  ( 30.90303789707364501, -285.1423027157269985, -239.1288291535903170 ) ) ;
#23898=CARTESIAN_POINT ( 'NONE',  ( -17.29563249692224147, -278.4477748599451843, -197.2963477405119477 ) ) ;
#23900=CARTESIAN_POINT ( 'NONE',  ( -84.90658679699598110, -283.2370646750198375, -325.8189397721372416 ) ) ;
#23901=CARTESIAN_POINT ( 'NONE',  ( -72.33916100788187009, -280.8045948323829748, -202.2056101964543302 ) ) ;
#23902=CARTESIAN_POINT ( 'NONE',  ( 25.35986498400079370, -286.0228087338464888, -226.0514999871602697 ) ) ;
#23903=CARTESIAN_POINT ( 'NONE',  ( -15.26955331896128598, -296.5227243923497440, -341.0605870371815627 ) ) ;
#23904=CARTESIAN_POINT ( 'NONE',  ( -99.79799510027925180, -279.5691221042563370, -314.0148879717900741 ) ) ;
#23905=CARTESIAN_POINT ( 'NONE',  ( -92.96387463440578358, -279.1447027761931849, -322.9677960686437928 ) ) ;
#23906=CARTESIAN_POINT ( 'NONE',  ( -64.33511580822029430, -277.2476619686501067, -338.2407217379158055 ) ) ;
#23907=CARTESIAN_POINT ( 'NONE',  ( -40.62323327122707894, -300.0109735787196428, -195.5869007918923330 ) ) ;
#23908=CARTESIAN_POINT ( 'NONE',  ( 20.08462882394540117, -284.8874804685262916, -222.3594286362373680 ) ) ;
#23909=CARTESIAN_POINT ( 'NONE',  ( -110.7656065109321872, -291.8942514084221784, -290.7417555607279382 ) ) ;
#23910=CARTESIAN_POINT ( 'NONE',  ( 24.68147399423603972, -293.0112072294700170, -309.5377965601114170 ) ) ;
#23912=CARTESIAN_POINT ( 'NONE',  ( 20.53736924031489863, -293.8454898468997953, -314.9023798082772601 ) ) ;
#23913=ORIENTED_EDGE ( 'NONE', *, *, #87263, .T. ) ;
#23914=CARTESIAN_POINT ( 'NONE',  ( -73.30099428914419946, -292.6663771704143642, -202.6083873396415242 ) ) ;
#23915=CARTESIAN_POINT ( 'NONE',  ( -27.55292716731614178, -280.8310658396268309, -197.8662740700175391 ) ) ;
#23917=CARTESIAN_POINT ( 'NONE',  ( -75.61367048977638206, -296.4746835240489986, -203.8415520073582456 ) ) ;
#23918=CARTESIAN_POINT ( 'NONE',  ( 22.00620840721034099, -287.5456827016009811, -221.4618486675311431 ) ) ;
#23919=CARTESIAN_POINT ( 'NONE',  ( 30.34612202740482445, -288.3610802007995630, -307.1346199572772662 ) ) ;
#23921=CARTESIAN_POINT ( 'NONE',  ( -95.13057066695022002, -284.2569086975846062, -315.0193357681693556 ) ) ;
#23922=CARTESIAN_POINT ( 'NONE',  ( 173.6393091186583035, 243.4999469645294425, -179.6212980618050210 ) ) ;
#23923=CARTESIAN_POINT ( 'NONE',  ( -114.0692606672204477, -271.5444964837377029, -270.3482881119212493 ) ) ;
#23924=CARTESIAN_POINT ( 'NONE',  ( -77.20900537737810509, -207.8186285356463259, -353.4261111359479060 ) ) ;
#23925=CARTESIAN_POINT ( 'NONE',  ( -27.00879002244773375, -276.1145696363147408, -342.7892388707338114 ) ) ;
#23926=CARTESIAN_POINT ( 'NONE',  ( -95.52671526393385193, -276.8477418197925886, -314.9562980829682601 ) ) ;
#23927=CARTESIAN_POINT ( 'NONE',  ( -73.93107113370481898, -273.2468667334241559, -202.5747474471526175 ) ) ;
#23928=CARTESIAN_POINT ( 'NONE',  ( -109.1284923609438238, -270.2178699211290791, -295.6185954890034964 ) ) ;
#23929=CARTESIAN_POINT ( 'NONE',  ( -94.85123006512304755, -276.5498030080088938, -320.8185479603513954 ) ) ;
#23930=CARTESIAN_POINT ( 'NONE',  ( -73.57003431435376228, -290.0391701915085605, -333.8223395237987461 ) ) ;
#23931=CARTESIAN_POINT ( 'NONE',  ( -9.194102113407405241, -299.1989826547440998, -193.5188644571881582 ) ) ;
#23932=CARTESIAN_POINT ( 'NONE',  ( -109.0745196346259007, -273.5566487964402427, -242.5068259347219168 ) ) ;
#23933=CARTESIAN_POINT ( 'NONE',  ( -109.7365167224504177, -296.8476136959104679, -260.5988440050695090 ) ) ;
#23936=CARTESIAN_POINT ( 'NONE',  ( -90.30196549952719920, -279.7140398929894332, -324.3280051383205773 ) ) ;
#23937=CARTESIAN_POINT ( 'NONE',  ( 19.73364297326644490, -281.7616661695618063, -322.0329710821996514 ) ) ;
#23938=CARTESIAN_POINT ( 'NONE',  ( -87.29616588362910079, -278.8482891705223778, -324.0153575546233355 ) ) ;
#23939=CARTESIAN_POINT ( 'NONE',  ( -108.6629507555766736, -280.6497591483076235, -243.9935703873790658 ) ) ;
#23940=CARTESIAN_POINT ( 'NONE',  ( 95.76662123053866083, -298.3250659313402480, -196.8050307037779021 ) ) ;
#23942=CARTESIAN_POINT ( 'NONE',  ( -6.771356966445523540, -280.6316374636527371, -204.0567934928062073 ) ) ;
#23943=CARTESIAN_POINT ( 'NONE',  ( 8.153700883368010466, -277.2507147900504378, -332.3489450671041254 ) ) ;
#23944=CARTESIAN_POINT ( 'NONE',  ( 34.58291505140212507, -277.8266213278472492, -291.6632550308056011 ) ) ;
#23945=CARTESIAN_POINT ( 'NONE',  ( 37.91497188685495701, -273.9592025254017926, -257.0560006027221789 ) ) ;
#23946=ORIENTED_EDGE ( 'NONE', *, *, #54972, .T. ) ;
#23948=CARTESIAN_POINT ( 'NONE',  ( -103.6984915610428288, -290.1643219826851805, -239.5491404876763113 ) ) ;
#23949=CARTESIAN_POINT ( 'NONE',  ( 0.2412273258851620195, -285.8876288778715775, -203.2578166836876221 ) ) ;
#23950=CARTESIAN_POINT ( 'NONE',  ( -33.46526014224244960, -281.2425783014975309, -344.2856181345452455 ) ) ;
#23951=CARTESIAN_POINT ( 'NONE',  ( 16.24255596435040161, -280.8479255910486359, -320.8737105092341722 ) ) ;
#23952=CARTESIAN_POINT ( 'NONE',  ( -95.81995174611536470, -291.9060327787839810, -317.3417518730313418 ) ) ;
#23953=CARTESIAN_POINT ( 'NONE',  ( -9.108713640866275441, -281.6348572780157156, -202.6113653671510804 ) ) ;
#23954=CARTESIAN_POINT ( 'NONE',  ( -82.35875606868249577, -271.4379707664899115, -210.3089252440176722 ) ) ;
#23955=CARTESIAN_POINT ( 'NONE',  ( -2.023218349699846375, -280.9922334229024727, -337.8818204526351110 ) ) ;
#23956=CARTESIAN_POINT ( 'NONE',  ( 3.169018264107629435, -296.5085695028729447, -333.5402786762712140 ) ) ;
#23957=CARTESIAN_POINT ( 'NONE',  ( -102.5305802070660803, -277.3091000817353802, -231.2154991483648985 ) ) ;
#23958=CARTESIAN_POINT ( 'NONE',  ( -74.05730758487722198, -278.2053778895952405, -333.5739081229071985 ) ) ;
#23959=CARTESIAN_POINT ( 'NONE',  ( -112.0782437926158082, -286.4494415202189543, -278.3909041774814455 ) ) ;
#23963=CARTESIAN_POINT ( 'NONE',  ( -107.0482918840414612, -292.8502531109541565, -241.2011237905825283 ) ) ;
#23964=CARTESIAN_POINT ( 'NONE',  ( 29.81017751619885559, -273.9942016173828279, -303.8791028315648646 ) ) ;
#23965=CARTESIAN_POINT ( 'NONE',  ( -48.85491922567549494, -288.3922638284930144, -346.3860276065843777 ) ) ;
#23966=CARTESIAN_POINT ( 'NONE',  ( -11.96620081880925035, -290.7877398135687486, -201.0063951513710663 ) ) ;
#23968=CARTESIAN_POINT ( 'NONE',  ( -107.5929501375299253, -276.9509359331373730, -292.1188166171854732 ) ) ;
#23969=CARTESIAN_POINT ( 'NONE',  ( -111.3324369047018649, -294.6057818723013497, -276.9867039834608704 ) ) ;
#23970=CARTESIAN_POINT ( 'NONE',  ( -94.47717563777250405, -291.2178609897763977, -316.5864456496148591 ) ) ;
#23973=CARTESIAN_POINT ( 'NONE',  ( 31.59526911869172494, -292.4565297260984948, -303.2012257864039384 ) ) ;
#23974=CARTESIAN_POINT ( 'NONE',  ( 36.35015695339029662, -289.0890404907353854, -265.5140760727286420 ) ) ;
#23975=CARTESIAN_POINT ( 'NONE',  ( -106.8141325011825984, -288.3924901878856986, -301.2730027581621925 ) ) ;
#23976=CARTESIAN_POINT ( 'NONE',  ( -44.09638606840582042, -287.3903494591515937, -197.0825458423149144 ) ) ;
#23978=CARTESIAN_POINT ( 'NONE',  ( 31.55489321480201781, -288.6819924654222405, -294.9753649245494671 ) ) ;
#23979=CARTESIAN_POINT ( 'NONE',  ( -71.30955064076870542, -297.4783258995264532, -337.6262050490568072 ) ) ;
#23982=CARTESIAN_POINT ( 'NONE',  ( 38.95768582296182103, -288.6644383284276500, -262.9801780157574740 ) ) ;
#23983=CARTESIAN_POINT ( 'NONE',  ( -31.18250303832461157, -278.1495677559947239, -195.2064831246659367 ) ) ;
#23984=CARTESIAN_POINT ( 'NONE',  ( -34.28768442688075879, -277.3480157702554152, -347.2793686106254540 ) ) ;
#23985=CARTESIAN_POINT ( 'NONE',  ( -16.99349426536716834, -279.9746637911981111, -196.1203285901392519 ) ) ;
#23986=CARTESIAN_POINT ( 'NONE',  ( -95.75385141253924814, -299.1738394472778282, -223.8867445098934468 ) ) ;
#23987=CARTESIAN_POINT ( 'NONE',  ( -94.77055790362604171, -283.2188027989268448, -222.1228868096299038 ) ) ;
#23989=CARTESIAN_POINT ( 'NONE',  ( -2.549558956960578548, -278.6569489036358505, -204.7694736121925416 ) ) ;
#23990=CARTESIAN_POINT ( 'NONE',  ( -106.3959287420960322, -282.1680181412125421, -299.7603465414932202 ) ) ;
#23992=CARTESIAN_POINT ( 'NONE',  ( -39.95873918027843530, -275.5643242329203417, -346.6358447972009458 ) ) ;
#23993=CARTESIAN_POINT ( 'NONE',  ( -104.5611745072759931, -297.6677642711055114, -300.6892603022994876 ) ) ;
#23994=CARTESIAN_POINT ( 'NONE',  ( -63.81825088255502010, -282.3097839389124033, -342.3367025211248347 ) ) ;
#23995=CARTESIAN_POINT ( 'NONE',  ( -97.08159317062981586, -298.0830161059922716, -227.9989458506799451 ) ) ;
#23996=CARTESIAN_POINT ( 'NONE',  ( -113.5943785400798731, -274.0489174888291473, -264.6882063956397246 ) ) ;
#23997=CARTESIAN_POINT ( 'NONE',  ( -8.958693874168883298, -274.1004872762172795, -203.0279766285698599 ) ) ;
#23998=CARTESIAN_POINT ( 'NONE',  ( 37.19753870975527832, -295.6647713107479944, -279.1194778449742557 ) ) ;
#23999=CARTESIAN_POINT ( 'NONE',  ( 21.49039423764156354, -288.3880808071408524, -320.0379201850865911 ) ) ;
#24000=CARTESIAN_POINT ( 'NONE',  ( -102.1634311530903432, -277.1491130150744198, -231.4334491674557341 ) ) ;
#24001=CARTESIAN_POINT ( 'NONE',  ( -114.3901496886219746, -290.3746479219313983, -271.2266388070503353 ) ) ;
#24002=CARTESIAN_POINT ( 'NONE',  ( -104.2676010946641441, -289.2103627284244567, -300.2241264792394873 ) ) ;
#24003=CARTESIAN_POINT ( 'NONE',  ( 36.10856825881999299, -291.3564332654094073, -255.1303845328275486 ) ) ;
#24005=CARTESIAN_POINT ( 'NONE',  ( 28.92138380700103895, -24.05900251067409457, -347.7894294321414463 ) ) ;
#24006=CARTESIAN_POINT ( 'NONE',  ( -102.4615737567793872, -290.5106841674224256, -237.1222601914937229 ) ) ;
#24008=CARTESIAN_POINT ( 'NONE',  ( -105.2296266693531237, -285.9587564480613082, -234.4136310133014263 ) ) ;
#24009=CARTESIAN_POINT ( 'NONE',  ( 13.13280560600884073, -291.7964315240021733, -212.5238939548889334 ) ) ;
#24010=CARTESIAN_POINT ( 'NONE',  ( 23.87067568443297816, -283.4820644124300770, -316.2560340571390611 ) ) ;
#24011=CARTESIAN_POINT ( 'NONE',  ( -103.0135927354892402, -283.9525244412004099, -302.3551481932249203 ) ) ;
#24012=CARTESIAN_POINT ( 'NONE',  ( -68.17745805382324420, -297.6584023455129682, -199.7482714480778725 ) ) ;
#24013=CARTESIAN_POINT ( 'NONE',  ( 11.86436072089016136, -276.0677416204142105, -215.7031678710926599 ) ) ;
#24014=CARTESIAN_POINT ( 'NONE',  ( -5.313529187195955572, -290.4957845859748886, -202.9226721014413783 ) ) ;
#24015=CARTESIAN_POINT ( 'NONE',  ( 19.31509798575756420, -273.6894139809560329, -223.7013094366977555 ) ) ;
#24018=CARTESIAN_POINT ( 'NONE',  ( -16.79747137322971184, -288.2395862551080086, -198.7583066653558603 ) ) ;
#24019=CARTESIAN_POINT ( 'NONE',  ( -114.0290016266300626, -297.6411369145560570, -269.6192974228089270 ) ) ;
#24020=CARTESIAN_POINT ( 'NONE',  ( -109.0305551328621902, -285.3919961689906586, -256.0572465978581818 ) ) ;
#24021=CARTESIAN_POINT ( 'NONE',  ( -113.8457029045860480, -277.5238828230081367, -277.2978523315670714 ) ) ;
#24022=CARTESIAN_POINT ( 'NONE',  ( 37.66004072891103505, -293.9903543095188638, -253.3300238259291177 ) ) ;
#24023=CARTESIAN_POINT ( 'NONE',  ( 24.82441493895079532, -286.2744659137090935, -313.7602766908942158 ) ) ;
#24024=CARTESIAN_POINT ( 'NONE',  ( 39.48135836021926082, -293.9563912595863258, -276.0333594785666378 ) ) ;
#24025=CARTESIAN_POINT ( 'NONE',  ( -36.21005868477442391, -292.3999731901431574, -197.3362630471475256 ) ) ;
#24026=DIRECTION ( 'NONE',  ( 1.000000000000000000, 0.000000000000000000, 0.000000000000000000 ) ) ;
#24028=CARTESIAN_POINT ( 'NONE',  ( -97.39219751933890734, -246.9239084015181902, -331.4851807666239552 ) ) ;
#24029=CARTESIAN_POINT ( 'NONE',  ( -113.5148738872261163, -286.0050369231415175, -275.6888339762146529 ) ) ;
#24030=CARTESIAN_POINT ( 'NONE',  ( -106.6379572354042296, -294.4809262143061233, -236.9535640164627353 ) ) ;
#24032=CARTESIAN_POINT ( 'NONE',  ( -53.77226634314865095, -282.1881939430227817, -341.8575472872119008 ) ) ;
#24033=CARTESIAN_POINT ( 'NONE',  ( -98.55696196329681413, -278.8414789833790906, -223.6659283124894841 ) ) ;
#24034=CARTESIAN_POINT ( 'NONE',  ( 29.40538630022882671, -283.1027979550383975, -236.4105907008620306 ) ) ;
#24035=CARTESIAN_POINT ( 'NONE',  ( -109.7673734041845250, -271.5244187881392577, -296.0454323531374712 ) ) ;
#24036=CARTESIAN_POINT ( 'NONE',  ( -74.00930885969619055, -282.1038073525274399, -337.4581557811464450 ) ) ;
#24037=CARTESIAN_POINT ( 'NONE',  ( 36.13644118953845918, -285.7418516898928260, -283.5068227219726964 ) ) ;
#24038=CARTESIAN_POINT ( 'NONE',  ( -78.19576668289161603, -275.3693793909611713, -206.5547646540406959 ) ) ;
#24039=CARTESIAN_POINT ( 'NONE',  ( -69.74572868557065419, -295.9831485914014024, -335.8436910468028032 ) ) ;
#24041=CARTESIAN_POINT ( 'NONE',  ( 13.25471663912096432, -291.4626902602138330, -217.0577776790478595 ) ) ;
#24042=CARTESIAN_POINT ( 'NONE',  ( -102.0067704589574902, -278.6557295953940070, -312.0724651775327629 ) ) ;
#24043=CARTESIAN_POINT ( 'NONE',  ( 5.396786294105012871, -276.4557763541437225, -329.6048022234635937 ) ) ;
#24044=CARTESIAN_POINT ( 'NONE',  ( -78.68652459779990238, -274.5887606757104891, -205.7693383287437996 ) ) ;
#24045=CARTESIAN_POINT ( 'NONE',  ( -103.3467885130483381, -276.9605693250397849, -309.5142434987732827 ) ) ;
#24046=CARTESIAN_POINT ( 'NONE',  ( 160.7988830095787876, 220.5294184113604103, -205.1624142897960041 ) ) ;
#24047=CARTESIAN_POINT ( 'NONE',  ( -83.93836615091302633, -275.6916119227558397, -329.1952503178288225 ) ) ;
#24048=CARTESIAN_POINT ( 'NONE',  ( 30.38850688036680125, -295.4372827684630920, -305.7337818621584802 ) ) ;
#24052=CARTESIAN_POINT ( 'NONE',  ( -108.3314206663945072, -285.8723084710375133, -252.0667021042178817 ) ) ;
#24053=CARTESIAN_POINT ( 'NONE',  ( -35.89570210073392786, -284.7944193386777556, -346.3469723819573005 ) ) ;
#24054=CARTESIAN_POINT ( 'NONE',  ( 9.101633486965683417, -286.0582559666873976, -213.9083994426079585 ) ) ;
#24055=CARTESIAN_POINT ( 'NONE',  ( 26.05247062488065524, -274.4658794630133229, -308.1449707306840651 ) ) ;
#24056=CARTESIAN_POINT ( 'NONE',  ( -21.09519838463042163, -284.7020652081021694, -342.8496178439958726 ) ) ;
#24057=CARTESIAN_POINT ( 'NONE',  ( -96.95528110235694896, -277.6326687465584655, -227.0375826116616906 ) ) ;
#24058=CARTESIAN_POINT ( 'NONE',  ( -8.604888092625166962, -277.7466936344683290, -337.8167068637942521 ) ) ;
#24060=CARTESIAN_POINT ( 'NONE',  ( -29.98990376932585633, -274.6400607751372149, -197.6704065268607735 ) ) ;
#24061=CARTESIAN_POINT ( 'NONE',  ( 24.45577590054008965, -281.7468264399373084, -224.6967907960918751 ) ) ;
#24062=CARTESIAN_POINT ( 'NONE',  ( 31.96330624505919360, -281.6141370065750493, -236.8268511722395715 ) ) ;
#24064=ORIENTED_EDGE ( 'NONE', *, *, #46511, .T. ) ;
#24066=CARTESIAN_POINT ( 'NONE',  ( 6.804669258927659392, -288.5056494202891599, -208.7221413189987516 ) ) ;
#24067=CARTESIAN_POINT ( 'NONE',  ( -90.15536508354232126, -296.4790531619310059, -219.6594025006754407 ) ) ;
#24068=CARTESIAN_POINT ( 'NONE',  ( -90.70921547136478580, -290.6682294340274098, -214.9227848401430094 ) ) ;
#24069=CARTESIAN_POINT ( 'NONE',  ( 34.68423810131464791, -286.2364437076421382, -286.0077860441973598 ) ) ;
#24070=CARTESIAN_POINT ( 'NONE',  ( -58.87877431507047277, -287.9108690292268875, -340.7814571186216881 ) ) ;
#24071=CARTESIAN_POINT ( 'NONE',  ( -33.23168645308187052, -287.3099947028100587, -197.0291167287993517 ) ) ;
#24072=CARTESIAN_POINT ( 'NONE',  ( -108.7699542241383739, -276.2548504244458627, -293.3978189630082625 ) ) ;
#24073=CARTESIAN_POINT ( 'NONE',  ( -38.92420283273519743, -287.4715737141797263, -346.5446864407430780 ) ) ;
#24074=CARTESIAN_POINT ( 'NONE',  ( -51.81299776773756349, -287.8672905748318271, -196.7174977352765097 ) ) ;
#24075=CARTESIAN_POINT ( 'NONE',  ( -62.18240498515375947, -287.3741381022549604, -341.3595797603300070 ) ) ;
#24076=CARTESIAN_POINT ( 'NONE',  ( 31.58009454605360844, -282.8239079437940404, -295.2738956358620612 ) ) ;
#24077=CARTESIAN_POINT ( 'NONE',  ( -63.76868395764510922, -293.7087111566713133, -199.9383623610897587 ) ) ;
#24081=CARTESIAN_POINT ( 'NONE',  ( -101.1143957367595902, -299.0135756114960373, -229.8351079163101076 ) ) ;
#24082=CARTESIAN_POINT ( 'NONE',  ( 9.387514357973238077, -279.9105285566134853, -214.0013558451431663 ) ) ;
#24083=CARTESIAN_POINT ( 'NONE',  ( 32.95352943092358089, -279.2108490648196835, -244.0665967520644415 ) ) ;
#24084=CARTESIAN_POINT ( 'NONE',  ( 27.96328084532138902, -293.2811028027144857, -310.9507902760603315 ) ) ;
#24085=CARTESIAN_POINT ( 'NONE',  ( -111.3550334602798841, -270.7922941965885570, -270.3387588715830248 ) ) ;
#24086=CARTESIAN_POINT ( 'NONE',  ( 37.08310203119101089, -273.6125308602656219, -268.8567847437584533 ) ) ;
#24087=CARTESIAN_POINT ( 'NONE',  ( -93.44810510923574043, -297.1969993751604306, -317.8497011250556170 ) ) ;
#24088=CARTESIAN_POINT ( 'NONE',  ( -109.5391439510883345, -271.4447933644419777, -245.3384203335399150 ) ) ;
#24089=CARTESIAN_POINT ( 'NONE',  ( -71.63701261007109622, -293.7388975568979959, -338.1682382464410352 ) ) ;
#24090=CARTESIAN_POINT ( 'NONE',  ( 15.28429262419472501, -294.2384285814295026, -218.8500356984787345 ) ) ;
#24092=CARTESIAN_POINT ( 'NONE',  ( 16.85092222879885071, -293.6515628917910021, -221.1364317592264968 ) ) ;
#24094=CARTESIAN_POINT ( 'NONE',  ( -111.3773302825175335, -282.7551080707198707, -256.0497324981460565 ) ) ;
#24095=CARTESIAN_POINT ( 'NONE',  ( -63.56899361707755958, -295.4036097707765975, -338.5405087687711330 ) ) ;
#24096=CARTESIAN_POINT ( 'NONE',  ( 23.40291776680545155, -282.1845285084945658, -317.7014633831005312 ) ) ;
#24097=CARTESIAN_POINT ( 'NONE',  ( 37.97436862015810277, -283.3949895945349340, -264.2944892374715664 ) ) ;
#24098=CARTESIAN_POINT ( 'NONE',  ( -30.88139700416046907, -285.7983820696040311, -193.6405339634017650 ) ) ;
#24099=CARTESIAN_POINT ( 'NONE',  ( -92.08334897910739869, -289.2679089808933668, -219.3188481302005641 ) ) ;
#24100=CARTESIAN_POINT ( 'NONE',  ( 37.98031237521716008, -280.1872657929903312, -282.6615398329582263 ) ) ;
#24101=CARTESIAN_POINT ( 'NONE',  ( 15.39495156249690488, -285.5019081419919758, -219.1743125896222466 ) ) ;
#24102=CARTESIAN_POINT ( 'NONE',  ( -3.210702582081981227, -287.5323454636259726, -339.0529575108198514 ) ) ;
#24104=CARTESIAN_POINT ( 'NONE',  ( -20.64761206647024849, -296.4345130589201176, -342.3008465266025269 ) ) ;
#24105=CARTESIAN_POINT ( 'NONE',  ( -102.9153380359032894, -280.4940004957827000, -231.0318765051935088 ) ) ;
#24106=CARTESIAN_POINT ( 'NONE',  ( -41.87242274252311347, -293.1289512496367706, -345.6312679145259494 ) ) ;
#24107=CARTESIAN_POINT ( 'NONE',  ( -41.04801483223821634, -279.6709406116780201, -197.4340947460692348 ) ) ;
#24108=CARTESIAN_POINT ( 'NONE',  ( 39.22589159581952600, -293.6108102615382904, -261.7238101312024696 ) ) ;
#24109=CARTESIAN_POINT ( 'NONE',  ( -49.09613425688456090, -283.9834865030073843, -195.6682691328664134 ) ) ;
#24110=CARTESIAN_POINT ( 'NONE',  ( -104.5417644539270299, -280.1114965846896894, -303.7818189914986533 ) ) ;
#24112=CARTESIAN_POINT ( 'NONE',  ( -71.04973375405431568, -294.5671396668164448, -335.3918917136205664 ) ) ;
#24113=CARTESIAN_POINT ( 'NONE',  ( -37.57518916095028061, -296.0490714493265045, -195.3614770738068387 ) ) ;
#24116=CARTESIAN_POINT ( 'NONE',  ( 23.94941473222153761, -284.1127613472592657, -312.9668223289573916 ) ) ;
#24117=CARTESIAN_POINT ( 'NONE',  ( -88.54944952712649808, -295.3015085682924337, -322.5451279973512442 ) ) ;
#24120=CARTESIAN_POINT ( 'NONE',  ( 35.78497577281001440, -278.8380690714489560, -253.7030783399848985 ) ) ;
#24121=CARTESIAN_POINT ( 'NONE',  ( -34.09975461072447445, -273.2891254431398238, -193.5910156633567567 ) ) ;
#24122=CARTESIAN_POINT ( 'NONE',  ( -8.404038286393724633, -289.9963363167768193, -341.1983837932966139 ) ) ;
#24123=CARTESIAN_POINT ( 'NONE',  ( -90.59421059806915366, -289.6662681520369347, -320.3665941199759573 ) ) ;
#24124=CARTESIAN_POINT ( 'NONE',  ( -8.998403965952357808, -281.9498526219713881, -202.3363775124014410 ) ) ;
#24125=CARTESIAN_POINT ( 'NONE',  ( -102.7488135132294644, -274.6137010119094839, -236.0692410952486568 ) ) ;
#24126=CARTESIAN_POINT ( 'NONE',  ( -57.20601436142635521, -278.5849814165087537, -199.7032130898164439 ) ) ;
#24128=CARTESIAN_POINT ( 'NONE',  ( -101.2073588118438323, -272.9532307374003608, -227.2525068493970082 ) ) ;
#24129=CARTESIAN_POINT ( 'NONE',  ( 3.000762344979050589, -294.5181086247619646, -207.7396978107178711 ) ) ;
#24131=CARTESIAN_POINT ( 'NONE',  ( -108.5286334908166737, -291.4232610434195294, -253.6838318876198457 ) ) ;
#24133=CARTESIAN_POINT ( 'NONE',  ( -58.56953896801237391, -289.9201061846744665, -197.6309018657443914 ) ) ;
#24134=CARTESIAN_POINT ( 'NONE',  ( -70.47334986065760631, -297.2695722315889952, -205.2750790525290654 ) ) ;
#24136=CARTESIAN_POINT ( 'NONE',  ( -98.65911243411574105, -292.6817630445017926, -224.9202536514419819 ) ) ;
#24137=CARTESIAN_POINT ( 'NONE',  ( -119.3990491898856732, -299.0519495502701943, -270.3937649182068412 ) ) ;
#24138=CARTESIAN_POINT ( 'NONE',  ( 37.09547970612607060, -289.4533585897438002, -262.6712100871828852 ) ) ;
#24139=CARTESIAN_POINT ( 'NONE',  ( 19.68949475164547280, -274.2240834885686240, -318.8118273691307536 ) ) ;
#24140=CARTESIAN_POINT ( 'NONE',  ( 3.703958444967716535, -276.5289197830974217, -208.1982527677516828 ) ) ;
#24141=CARTESIAN_POINT ( 'NONE',  ( 17.82142236992688922, -290.9290158271220434, -220.3020482852665509 ) ) ;
#24142=CARTESIAN_POINT ( 'NONE',  ( -71.96384143193522220, -281.4598290435216654, -202.9552106530227604 ) ) ;
#24144=CARTESIAN_POINT ( 'NONE',  ( 33.05537322495047903, -281.1607716488837241, -290.0625070634780514 ) ) ;
#24145=CARTESIAN_POINT ( 'NONE',  ( -54.05045401314183806, -278.3413657381316852, -345.2641178048867800 ) ) ;
#24146=CARTESIAN_POINT ( 'NONE',  ( -3.084253864379969734, -281.4046670687133656, -338.8916495060582292 ) ) ;
#24147=CARTESIAN_POINT ( 'NONE',  ( -64.99907447057177023, -278.3458907325305063, -342.0265140400529731 ) ) ;
#24149=CARTESIAN_POINT ( 'NONE',  ( -52.42766400724116238, -275.3825835483822289, -195.5066199320201008 ) ) ;
#24150=CARTESIAN_POINT ( 'NONE',  ( -82.08285599513421005, -280.1948066931273615, -326.5171145203363494 ) ) ;
#24153=CARTESIAN_POINT ( 'NONE',  ( -111.1046351201329969, -298.3772169364756905, -283.9979007281625627 ) ) ;
#24154=CARTESIAN_POINT ( 'NONE',  ( -37.25390324154415111, -290.1307009779644659, -343.6701785853040860 ) ) ;
#24155=CARTESIAN_POINT ( 'NONE',  ( 5.011349368260566095, -290.2482910822479312, -333.4498904414700746 ) ) ;
#24156=CARTESIAN_POINT ( 'NONE',  ( -32.14176661739875840, -291.4680244683075330, -197.4317236692579343 ) ) ;
#24157=CARTESIAN_POINT ( 'NONE',  ( 38.61320028161129159, -287.2173468159307959, -282.9478121757559279 ) ) ;
#24159=CARTESIAN_POINT ( 'NONE',  ( -101.1024427810556148, -282.4475416280000104, -307.5230354533509285 ) ) ;
#24160=CARTESIAN_POINT ( 'NONE',  ( -111.5719011644520862, -292.4013956106432488, -271.2229367236711823 ) ) ;
#24161=CARTESIAN_POINT ( 'NONE',  ( -94.64910958572320965, -283.6813277305129191, -224.0100495101620481 ) ) ;
#24162=CARTESIAN_POINT ( 'NONE',  ( -19.43047097031776715, -281.6024504666851840, -199.0313334681027300 ) ) ;
#24163=CARTESIAN_POINT ( 'NONE',  ( -3.154718925215548531, -289.5529418247576814, -339.1075769570591092 ) ) ;
#24164=CARTESIAN_POINT ( 'NONE',  ( -109.6836514192032155, -279.1839540675258036, -259.7809594759498282 ) ) ;
#24165=CARTESIAN_POINT ( 'NONE',  ( -73.23401242778071207, -290.3819992879446659, -202.6724414925973292 ) ) ;
#24166=CARTESIAN_POINT ( 'NONE',  ( 5.081986803286600463, -287.4124233823784493, -206.2322390820201292 ) ) ;
#24167=CARTESIAN_POINT ( 'NONE',  ( -97.53617769424801054, -285.6865395604866080, -222.4429400733428963 ) ) ;
#24168=CARTESIAN_POINT ( 'NONE',  ( -69.00724396369996327, -283.6472497812994789, -336.1494852067335728 ) ) ;
#24171=CARTESIAN_POINT ( 'NONE',  ( -19.69779548106202682, -294.1369444681128584, -196.6254443763347979 ) ) ;
#24172=CARTESIAN_POINT ( 'NONE',  ( 39.16350184510627486, -292.2006147227178872, -267.4720409403039980 ) ) ;
#24173=CARTESIAN_POINT ( 'NONE',  ( -41.88311313187436014, -276.1694909777545490, -343.4681050640111266 ) ) ;
#24175=CARTESIAN_POINT ( 'NONE',  ( -60.10998323911704233, -297.1133091972114357, -196.8555655907056803 ) ) ;
#24177=CARTESIAN_POINT ( 'NONE',  ( 32.46398070410751302, -291.7192834577892881, -246.5827713165533339 ) ) ;
#24178=CARTESIAN_POINT ( 'NONE',  ( -78.05088637139978403, -295.7369702212350830, -208.4874396830663272 ) ) ;
#24179=CARTESIAN_POINT ( 'NONE',  ( -92.86688826628117965, -292.4374696092740464, -222.3602431167188911 ) ) ;
#24180=CARTESIAN_POINT ( 'NONE',  ( 22.04708407315842322, -294.0328264091616575, -227.3607306866663293 ) ) ;
#24182=CARTESIAN_POINT ( 'NONE',  ( 16.23645552972213224, -292.2941826334723601, -323.1552297913313510 ) ) ;
#24184=CARTESIAN_POINT ( 'NONE',  ( -112.3201108662026400, -298.5947487997715939, -267.0564237451849294 ) ) ;
#24185=CARTESIAN_POINT ( 'NONE',  ( 35.91539534603148809, -288.4662274997117493, -268.2938975531151300 ) ) ;
#24186=CARTESIAN_POINT ( 'NONE',  ( 21.37558129910982174, -278.1790031429999317, -317.6116938469855882 ) ) ;
#24187=CARTESIAN_POINT ( 'NONE',  ( -88.95595053112002404, -276.5535686918682359, -326.9648093196621517 ) ) ;
#24188=CARTESIAN_POINT ( 'NONE',  ( -38.34774694635147796, -273.3884413390801456, -193.4696317380877133 ) ) ;
#24189=CARTESIAN_POINT ( 'NONE',  ( 34.85812525177245647, -279.3968261568018647, -252.1847070104660702 ) ) ;
#24190=CARTESIAN_POINT ( 'NONE',  ( -38.55289252647968112, -275.4669799786212252, -346.5514942191414889 ) ) ;
#24192=CARTESIAN_POINT ( 'NONE',  ( -82.67709312739731331, -294.3711659101185205, -328.2701625731981494 ) ) ;
#24193=CARTESIAN_POINT ( 'NONE',  ( -75.83866562722688798, -275.5387618305366573, -205.9355391194186780 ) ) ;
#24194=CARTESIAN_POINT ( 'NONE',  ( -34.48223376678599550, -298.8916831039321664, -197.1992380068014370 ) ) ;
#24196=CARTESIAN_POINT ( 'NONE',  ( -94.23343959948523718, -287.8898220745959406, -319.7750510876022076 ) ) ;
#24197=CARTESIAN_POINT ( 'NONE',  ( 31.11905179698761259, -275.0475697052659712, -245.0209236197029554 ) ) ;
#24198=CARTESIAN_POINT ( 'NONE',  ( 38.67497842921257245, -287.7096145223900407, -282.9516801271768713 ) ) ;
#24199=CARTESIAN_POINT ( 'NONE',  ( -108.3778075964839189, -274.8696739443033721, -245.7867439049370546 ) ) ;
#24200=CARTESIAN_POINT ( 'NONE',  ( -83.51042277272051706, -293.6862896706013544, -329.3209835028397379 ) ) ;
#24201=CARTESIAN_POINT ( 'NONE',  ( -83.79373517715774256, -282.8685375476570698, -331.6355378381636001 ) ) ;
#24203=CARTESIAN_POINT ( 'NONE',  ( 35.74198568589435610, -279.3350511499395452, -253.4595420684386795 ) ) ;
#24205=CARTESIAN_POINT ( 'NONE',  ( -100.6541973942827042, -288.8388165928553803, -307.5915418789282967 ) ) ;
#24206=CARTESIAN_POINT ( 'NONE',  ( -100.0875395593015469, -282.1515326856607544, -310.1288638457169782 ) ) ;
#24210=CARTESIAN_POINT ( 'NONE',  ( -111.6068545495161146, -288.4163302950433376, -280.9266537294239470 ) ) ;
#24211=CARTESIAN_POINT ( 'NONE',  ( -74.64086251223216095, -275.0666614153669229, -206.7450917909235102 ) ) ;
#24212=CARTESIAN_POINT ( 'NONE',  ( -30.23636762041420312, -284.1692178395238102, -346.6338062024674400 ) ) ;
#24213=CARTESIAN_POINT ( 'NONE',  ( -64.36186634220776170, -271.7821386223063200, -199.7835771281365567 ) ) ;
#24214=CARTESIAN_POINT ( 'NONE',  ( -73.79679229502430360, -283.5503328884254870, -333.6644825090182849 ) ) ;
#24215=CARTESIAN_POINT ( 'NONE',  ( 35.20348540882881849, -276.8148124321920136, -257.9344166695875629 ) ) ;
#24216=CARTESIAN_POINT ( 'NONE',  ( 28.17966191647327889, -276.7967436675832573, -303.0261309458548453 ) ) ;
#24217=CARTESIAN_POINT ( 'NONE',  ( 1.091704864048238521, -284.5392268195603265, -334.7651087697895491 ) ) ;
#24219=DIRECTION ( 'NONE',  ( 0.9999189529070979798, -0.01273136352371030157, 0.000000000000000000 ) ) ;
#24220=CARTESIAN_POINT ( 'NONE',  ( -114.3662701192796902, -296.3591270630996064, -272.4676747528282021 ) ) ;
#24221=CARTESIAN_POINT ( 'NONE',  ( 30.28981536891485504, -289.1148842548566336, -238.7727512765025608 ) ) ;
#24223=CARTESIAN_POINT ( 'NONE',  ( 44.71564893372296723, -291.0523547857347353, -270.3937649182068412 ) ) ;
#24224=CARTESIAN_POINT ( 'NONE',  ( -50.87153719638330784, -278.8034896274349421, -194.8731320652599948 ) ) ;
#24225=CARTESIAN_POINT ( 'NONE',  ( -40.57783604249069498, -290.4120001036104668, -194.2168185693909379 ) ) ;
#24226=CARTESIAN_POINT ( 'NONE',  ( -109.3464679038811340, -286.2780121446183443, -254.6170723644917757 ) ) ;
#24227=CARTESIAN_POINT ( 'NONE',  ( -54.75261396379869439, -281.5855864304346596, -198.3718723131606794 ) ) ;
#24228=CARTESIAN_POINT ( 'NONE',  ( -104.9195258151892887, -286.4426988563691339, -234.5848582629495525 ) ) ;
#24229=CARTESIAN_POINT ( 'NONE',  ( 19.12703919101086569, -284.2377290810115369, -319.7198267435823027 ) ) ;
#24230=CARTESIAN_POINT ( 'NONE',  ( 35.20168651080174982, -276.0464200419949066, -296.3341210845319438 ) ) ;
#24231=CARTESIAN_POINT ( 'NONE',  ( -109.7065170970319627, -270.7998507873303424, -251.1006153585047969 ) ) ;
#24232=CARTESIAN_POINT ( 'NONE',  ( -108.5118480687430065, -278.7590219587250431, -240.9704724198646204 ) ) ;
#24233=CARTESIAN_POINT ( 'NONE',  ( -89.14507455184212859, -299.2372652091091823, -216.8314382558901343 ) ) ;
#24235=CARTESIAN_POINT ( 'NONE',  ( -54.49178911615187815, -282.3376638359844719, -195.3683826091709363 ) ) ;
#24237=CARTESIAN_POINT ( 'NONE',  ( -54.29536025777959907, -295.9762185724656547, -196.5175069794742342 ) ) ;
#24240=CARTESIAN_POINT ( 'NONE',  ( -68.06900606460516201, -276.9744843056770947, -336.6607821356309955 ) ) ;
#24241=CARTESIAN_POINT ( 'NONE',  ( -1.500932584042229401, -275.7217004739361528, -202.6599503314498349 ) ) ;
#24243=CARTESIAN_POINT ( 'NONE',  ( 21.42214121125835646, -281.2780248760547579, -319.7537405569395332 ) ) ;
#24244=CARTESIAN_POINT ( 'NONE',  ( 25.10518689917867974, -289.8540604609663092, -310.0897010612146687 ) ) ;
#24245=CARTESIAN_POINT ( 'NONE',  ( -111.9233616223406926, -297.8686651190229213, -286.4944227929585168 ) ) ;
#24246=CARTESIAN_POINT ( 'NONE',  ( -112.2137909009417740, -297.5536698762014112, -286.5530525055098678 ) ) ;
#24247=CARTESIAN_POINT ( 'NONE',  ( -60.85868035426064893, -293.7465757129684221, -199.2646379196514488 ) ) ;
#24248=CARTESIAN_POINT ( 'NONE',  ( -1.574256382571885382, -280.5767895285446798, -336.1079355108132063 ) ) ;
#24249=CARTESIAN_POINT ( 'NONE',  ( -7.443080109860269467, -282.3673964200521027, -202.1754339639073521 ) ) ;
#24250=CARTESIAN_POINT ( 'NONE',  ( -94.70793355536595470, -295.2917258644264393, -222.9026038185263587 ) ) ;
#24251=CARTESIAN_POINT ( 'NONE',  ( -96.96728401389962926, -286.7941413610985251, -222.9139877716735612 ) ) ;
#24252=CARTESIAN_POINT ( 'NONE',  ( 33.37644657516987223, -286.7288443741358606, -289.8669640452080785 ) ) ;
#24253=CARTESIAN_POINT ( 'NONE',  ( 204.9738417247596658, 294.2970692423710375, -68.59889679756817316 ) ) ;
#24255=CARTESIAN_POINT ( 'NONE',  ( 25.35773390008506922, -286.7095393058192485, -314.1255814434051103 ) ) ;
#24256=CARTESIAN_POINT ( 'NONE',  ( 31.86198634145748798, -286.9094217880578981, -247.0601037174077703 ) ) ;
#24258=CARTESIAN_POINT ( 'NONE',  ( -10.79607422713366738, -283.7937614361280794, -342.3676783022263521 ) ) ;
#24259=CARTESIAN_POINT ( 'NONE',  ( 34.18613133314459418, -276.0791910466108448, -285.0531843216789980 ) ) ;
#24260=CARTESIAN_POINT ( 'NONE',  ( -40.60544878184765594, -290.9323729833776611, -193.7265787106126425 ) ) ;
#24261=CARTESIAN_POINT ( 'NONE',  ( 39.60839370530543846, -282.1980721830683478, -269.9225583204415102 ) ) ;
#24262=CARTESIAN_POINT ( 'NONE',  ( -11.76019300876496132, -281.8992612281266474, -198.4147965194464973 ) ) ;
#24263=CARTESIAN_POINT ( 'NONE',  ( 26.70664902961420850, -282.4476660923110671, -313.0642005608113436 ) ) ;
#24264=CARTESIAN_POINT ( 'NONE',  ( -19.53455508040201138, -280.2874880685394032, -199.5140147040914940 ) ) ;
#24265=CARTESIAN_POINT ( 'NONE',  ( -95.99890600148557951, -275.4094976428775681, -317.0979686699210447 ) ) ;
#24266=CARTESIAN_POINT ( 'NONE',  ( 161.9590788367351024, 220.0586530115249673, -205.3424623035032539 ) ) ;
#24268=CARTESIAN_POINT ( 'NONE',  ( 28.23101078672630493, -277.0705438268601597, -234.1942328955582298 ) ) ;
#24269=CARTESIAN_POINT ( 'NONE',  ( -100.5620283310121010, -247.3436685628221312, -333.7792060084481136 ) ) ;
#24270=CARTESIAN_POINT ( 'NONE',  ( 19.22715532734573074, -278.8937998667427678, -221.6402424963064846 ) ) ;
#24271=CARTESIAN_POINT ( 'NONE',  ( -33.79758114230445187, -297.4462576118440893, -197.2595890160661440 ) ) ;
#24272=CARTESIAN_POINT ( 'NONE',  ( 6.466340202544196281, -292.1377740889748793, -207.1125408801742367 ) ) ;
#24273=CARTESIAN_POINT ( 'NONE',  ( 103.6749136203638813, 114.2737147223544980, -279.7089131145189640 ) ) ;
#24274=CARTESIAN_POINT ( 'NONE',  ( -95.11359383969195846, -295.8083714035957996, -220.2720288792392580 ) ) ;
#24275=CARTESIAN_POINT ( 'NONE',  ( -102.3574731148658685, -288.4797317077532739, -305.3892826583979740 ) ) ;
#24276=CARTESIAN_POINT ( 'NONE',  ( -109.1586195450475287, -298.1679774236464482, -289.2048122262592074 ) ) ;
#24277=CARTESIAN_POINT ( 'NONE',  ( 26.78958423513960341, -288.3783803064957283, -234.3624424061470677 ) ) ;
#24279=CARTESIAN_POINT ( 'NONE',  ( 17.31363320724381083, -293.7501166772028114, -216.3825256813565545 ) ) ;
#24280=CARTESIAN_POINT ( 'NONE',  ( -93.30627762578858153, -285.7109073314539955, -223.3935280152225289 ) ) ;
#24281=CARTESIAN_POINT ( 'NONE',  ( -77.97875646948075712, -296.3137849303000166, -205.4254700686850299 ) ) ;
#24282=CARTESIAN_POINT ( 'NONE',  ( -13.92541250117955443, -293.1511306104014238, -197.1216835612295313 ) ) ;
#24283=CARTESIAN_POINT ( 'NONE',  ( 11.07519197877918771, -293.1939908009152873, -210.4985030882643287 ) ) ;
#24284=CARTESIAN_POINT ( 'NONE',  ( -26.47279292304417808, -289.0768105271383774, -342.5985018234167114 ) ) ;
#24285=ORIENTED_EDGE ( 'NONE', *, *, #54972, .F. ) ;
#24287=CARTESIAN_POINT ( 'NONE',  ( -36.58036543080844893, -299.9219959840034448, -194.5960722939407788 ) ) ;
#24288=CARTESIAN_POINT ( 'NONE',  ( -92.87368841189365298, -272.0721504827067747, -217.5763947807699594 ) ) ;
#24289=CARTESIAN_POINT ( 'NONE',  ( 33.18280814012359770, -280.8709796995106558, -290.1019939021576874 ) ) ;
#24292=CARTESIAN_POINT ( 'NONE',  ( -82.51521924894002780, -277.1586896621950586, -332.6417736735991184 ) ) ;
#24293=CARTESIAN_POINT ( 'NONE',  ( -110.6784991410187757, -271.0597417575163490, -262.1055547055786406 ) ) ;
#24294=CARTESIAN_POINT ( 'NONE',  ( -111.5873350432268722, -280.4446259531778196, -267.8903948359456990 ) ) ;
#24295=CARTESIAN_POINT ( 'NONE',  ( 12.56080270789499487, -274.4878402604188636, -325.3908880768925656 ) ) ;
#24296=CARTESIAN_POINT ( 'NONE',  ( -98.78835777911763216, -298.3116221860647101, -230.1263875913131187 ) ) ;
#24297=CARTESIAN_POINT ( 'NONE',  ( -103.4225237095337206, -273.9189986462070010, -238.7900362436460000 ) ) ;
#24298=CARTESIAN_POINT ( 'NONE',  ( -62.59928861108281239, -299.3289698360263174, -198.4688747391317634 ) ) ;
#24299=CARTESIAN_POINT ( 'NONE',  ( 6.303319244628854179, -272.6612211715428771, -208.8680902416132596 ) ) ;
#24300=CARTESIAN_POINT ( 'NONE',  ( 29.94632766610666508, -293.8189749331306757, -241.6621893811352777 ) ) ;
#24301=CARTESIAN_POINT ( 'NONE',  ( -37.53340930219462024, -290.6244680464102998, -196.7595922293898525 ) ) ;
#24303=CARTESIAN_POINT ( 'NONE',  ( -74.06195589420678971, -278.0189512674766092, -337.9863856052576239 ) ) ;
#24304=CARTESIAN_POINT ( 'NONE',  ( 51.69745723989969832, -299.5303143563324966, -197.3348114162781428 ) ) ;
#24305=CARTESIAN_POINT ( 'NONE',  ( -1.877699816360418383, -281.2771417231817850, -338.1519946243802792 ) ) ;
#24306=CARTESIAN_POINT ( 'NONE',  ( -64.90689019827060235, -297.4114969678361717, -340.3048835006177910 ) ) ;
#24308=CARTESIAN_POINT ( 'NONE',  ( -76.22157757107966347, -282.7831746026973860, -332.3964905384666508 ) ) ;
#24309=CARTESIAN_POINT ( 'NONE',  ( -84.96106770288503185, -281.7072597180340949, -328.5197308893282866 ) ) ;
#24311=CARTESIAN_POINT ( 'NONE',  ( 30.72670629406963627, -273.7534867197089170, -242.2617713174311689 ) ) ;
#24312=CARTESIAN_POINT ( 'NONE',  ( 21.43851144482888316, -282.9121620262820898, -223.7588380462409816 ) ) ;
#24313=DIRECTION ( 'NONE',  ( 0.000000000000000000, 0.000000000000000000, -1.000000000000000000 ) ) ;
#24315=CARTESIAN_POINT ( 'NONE',  ( -98.90851247555033865, -271.5552406034108799, -225.3741209302029347 ) ) ;
#24317=CARTESIAN_POINT ( 'NONE',  ( -42.65064294726608551, -279.1191573723599504, -345.3400720521835296 ) ) ;
#24319=CARTESIAN_POINT ( 'NONE',  ( -51.91986632276809388, -287.7872970238780113, -196.1673931677192968 ) ) ;
#24321=CARTESIAN_POINT ( 'NONE',  ( -111.8195757655022362, -288.4331562028644385, -279.6161404091726581 ) ) ;
#24323=CARTESIAN_POINT ( 'NONE',  ( -97.19771252494237501, -295.9370350467070239, -227.8830261546357008 ) ) ;
#24324=CARTESIAN_POINT ( 'NONE',  ( 18.74342339430308613, -286.3740383488456018, -319.0726523023352001 ) ) ;
#24325=CARTESIAN_POINT ( 'NONE',  ( -104.1716275211822733, -250.7505522545870349, -322.2422935457555582 ) ) ;
#24326=CARTESIAN_POINT ( 'NONE',  ( -110.1093869337224476, -294.7858889324204483, -252.1464442234635044 ) ) ;
#24327=CARTESIAN_POINT ( 'NONE',  ( 38.91045972137419540, -286.0830735237381646, -274.4056629616819123 ) ) ;
#24328=CARTESIAN_POINT ( 'NONE',  ( 35.49638471936595607, -283.3072586647704725, -282.2377257329421809 ) ) ;
#24329=CARTESIAN_POINT ( 'NONE',  ( -58.22999750475583625, -281.5581957003898310, -343.4751341312302770 ) ) ;
#24330=CARTESIAN_POINT ( 'NONE',  ( -52.36976945815977302, -291.8544398752798656, -198.8728319199562691 ) ) ;
#24331=CARTESIAN_POINT ( 'NONE',  ( 35.61450675344872963, -282.8464425558232165, -260.3514056018166229 ) ) ;
#24332=CARTESIAN_POINT ( 'NONE',  ( 35.30138319815173986, -282.4748614151007473, -279.4682145734781784 ) ) ;
#24333=CARTESIAN_POINT ( 'NONE',  ( 32.32887229441965360, -289.1576213026174855, -241.5122298157696434 ) ) ;
#24334=CARTESIAN_POINT ( 'NONE',  ( -102.7033263310560613, -273.4175613933858813, -229.6966112035494518 ) ) ;
#24337=CARTESIAN_POINT ( 'NONE',  ( -15.39432758174546834, -286.8502131026759230, -342.7181516561406056 ) ) ;
#24338=CARTESIAN_POINT ( 'NONE',  ( 34.72175344733467739, -275.2089597335130406, -243.2344031283086849 ) ) ;
#24339=CARTESIAN_POINT ( 'NONE',  ( 5.425844954331937586, -294.6136720717660751, -209.1194750718689761 ) ) ;
#24341=CARTESIAN_POINT ( 'NONE',  ( 39.58706461736021254, -284.0519495502703080, -270.3284710469133074 ) ) ;
#24342=CARTESIAN_POINT ( 'NONE',  ( -9.905297844479640901, -274.6945206840613309, -340.3416313900506225 ) ) ;
#24344=CARTESIAN_POINT ( 'NONE',  ( -99.25948310422523946, -295.5467948971788701, -225.9468346075454406 ) ) ;
#24345=CARTESIAN_POINT ( 'NONE',  ( -73.03150804686684694, -293.1713289379279104, -205.7074153091119513 ) ) ;
#24346=CARTESIAN_POINT ( 'NONE',  ( -46.18289457702470457, -273.2856150381182943, -197.7957960390364462 ) ) ;
#24347=CARTESIAN_POINT ( 'NONE',  ( -91.08525879867467268, -291.3527980317498418, -320.8572153504027824 ) ) ;
#24348=CARTESIAN_POINT ( 'NONE',  ( -91.85629734562050430, -292.1911997559498673, -221.4387056104807812 ) ) ;
#24349=CARTESIAN_POINT ( 'NONE',  ( -100.4853845514942776, -286.8381779065268233, -231.6519090120511066 ) ) ;
#24350=CARTESIAN_POINT ( 'NONE',  ( -36.40397259429063581, -293.4889587330746394, -193.9431664607276673 ) ) ;
#24351=CARTESIAN_POINT ( 'NONE',  ( -8.711406675527110011, -293.7342261557831193, -199.4132175916119536 ) ) ;
#24352=CARTESIAN_POINT ( 'NONE',  ( -45.09284468568896642, -294.9862212372054842, -342.9989198077045103 ) ) ;
#24353=CARTESIAN_POINT ( 'NONE',  ( 21.08719573798560276, -290.1993422423867059, -317.3830786111255406 ) ) ;
#24354=CARTESIAN_POINT ( 'NONE',  ( 38.25428318341963063, -281.5357731262338916, -255.7239286454167200 ) ) ;
#24355=CARTESIAN_POINT ( 'NONE',  ( -94.46608116275987754, -295.3135696117554971, -220.8248032016122977 ) ) ;
#24356=CARTESIAN_POINT ( 'NONE',  ( -113.1373569456931847, -284.2121577861798869, -284.2192529820676441 ) ) ;
#24357=CARTESIAN_POINT ( 'NONE',  ( 8.612400029370858690, -278.3993572042601272, -329.2493368985307711 ) ) ;
#24358=CARTESIAN_POINT ( 'NONE',  ( -95.44011067312165153, -282.7188007381790840, -315.2336758597690505 ) ) ;
#24359=CARTESIAN_POINT ( 'NONE',  ( 34.85213977616518832, -285.8140253508835826, -290.7317924749037275 ) ) ;
#24360=CARTESIAN_POINT ( 'NONE',  ( -20.42531841213682142, -274.9768567483539528, -344.2671146811232461 ) ) ;
#24362=CARTESIAN_POINT ( 'NONE',  ( -64.08372878085729951, -282.9183100446239791, -338.3526788209623533 ) ) ;
#24363=CARTESIAN_POINT ( 'NONE',  ( -67.22180021340106748, -280.8740381786061562, -199.8261030034607302 ) ) ;
#24364=CARTESIAN_POINT ( 'NONE',  ( 16.51231838533912821, -287.3683010807159235, -325.1393639240641846 ) ) ;
#24365=CARTESIAN_POINT ( 'NONE',  ( 15.04920196383539910, -296.0611896813401245, -322.7129060200044250 ) ) ;
#24366=CARTESIAN_POINT ( 'NONE',  ( 31.81832029625696734, -276.7372646615794451, -238.2459767620450179 ) ) ;
#24367=CARTESIAN_POINT ( 'NONE',  ( -5.335921001910500117, -275.7797282813993434, -200.8706267114634159 ) ) ;
#24368=CARTESIAN_POINT ( 'NONE',  ( -85.10684501570408145, -277.5663644770924634, -325.6321643212310732 ) ) ;
#24369=CARTESIAN_POINT ( 'NONE',  ( -103.4996737246296306, -274.9934036946292508, -235.6807659431107709 ) ) ;
#24370=CARTESIAN_POINT ( 'NONE',  ( 36.56595996537395621, -285.7040377118107699, -282.1765833907036267 ) ) ;
#24371=CARTESIAN_POINT ( 'NONE',  ( -111.4795524898663501, -291.9290519155388210, -288.0242503932797149 ) ) ;
#24372=CARTESIAN_POINT ( 'NONE',  ( -58.51058166895605694, -294.2527064381346236, -340.5473312100658632 ) ) ;
#24374=CARTESIAN_POINT ( 'NONE',  ( -65.33114033562596035, -291.3426767237926924, -202.9037071871791227 ) ) ;
#24376=CARTESIAN_POINT ( 'NONE',  ( -5.741253553265432963, -289.7259302266780310, -340.2388990512517921 ) ) ;
#24377=CARTESIAN_POINT ( 'NONE',  ( -94.02481673644157922, -279.8560606211833601, -224.1992618660642336 ) ) ;
#24379=CARTESIAN_POINT ( 'NONE',  ( -114.0000852372007785, -295.5180006597656757, -266.7361233282131820 ) ) ;
#24380=CARTESIAN_POINT ( 'NONE',  ( 12.35627453661135178, -289.0322970860686382, -329.0418141313459159 ) ) ;
#24381=CARTESIAN_POINT ( 'NONE',  ( -26.62824829141964855, -286.5180321343456171, -194.0779399989860394 ) ) ;
#24382=CARTESIAN_POINT ( 'NONE',  ( -102.2591279873634136, -285.3398042651627406, -236.9273768395715365 ) ) ;
#24383=CARTESIAN_POINT ( 'NONE',  ( 138.6955843366410477, 180.6821896333715642, -241.4130191322238090 ) ) ;
#24384=CARTESIAN_POINT ( 'NONE',  ( -14.30945429173846861, -91.08059216271270486, -358.4537093730789934 ) ) ;
#24385=CARTESIAN_POINT ( 'NONE',  ( 102.5375343959159409, 114.7846795236941801, -279.4961139801552008 ) ) ;
#24387=CARTESIAN_POINT ( 'NONE',  ( -96.22904551800844786, -277.1419397117301173, -313.7973516018416262 ) ) ;
#24388=CARTESIAN_POINT ( 'NONE',  ( -73.00435616091196778, -276.4568957866198957, -334.4255505339396564 ) ) ;
#24389=CARTESIAN_POINT ( 'NONE',  ( -81.23484655183182213, -273.1404642512579812, -207.0578043764131166 ) ) ;
#24390=CARTESIAN_POINT ( 'NONE',  ( -81.50421288696699662, -219.8904477667203423, -350.0058313318409091 ) ) ;
#24391=CARTESIAN_POINT ( 'NONE',  ( -20.25265699324641488, -275.5220109419201435, -344.9893587204326195 ) ) ;
#24393=CARTESIAN_POINT ( 'NONE',  ( -98.89023426883694867, -290.5004214998705834, -309.7281903496019027 ) ) ;
#24394=CARTESIAN_POINT ( 'NONE',  ( -26.24898243239163165, -298.9905479402500532, -193.5211247304686424 ) ) ;
#24395=CARTESIAN_POINT ( 'NONE',  ( 34.48149372902969390, -286.0328558528602798, -254.7831751228318922 ) ) ;
#24396=CARTESIAN_POINT ( 'NONE',  ( -112.9695772163608609, -273.3814310284679436, -256.1577181962400118 ) ) ;
#24397=CARTESIAN_POINT ( 'NONE',  ( -0.7561117800409273837, -294.7186870207760307, -333.5891748917225073 ) ) ;
#24399=CARTESIAN_POINT ( 'NONE',  ( -9.715114130673581982, -278.6142025350492872, -340.6895328978299631 ) ) ;
#24400=CARTESIAN_POINT ( 'NONE',  ( 38.08397996782814943, -281.2498314348806616, -285.5431364755187360 ) ) ;
#24401=CARTESIAN_POINT ( 'NONE',  ( -77.00059252077886640, -280.5871340552306492, -208.6451161851530287 ) ) ;
#24402=CARTESIAN_POINT ( 'NONE',  ( -64.70890802028478106, -279.1646478538789324, -341.3039601053520187 ) ) ;
#24403=CARTESIAN_POINT ( 'NONE',  ( -55.42100330385038376, -296.3898035015602090, -198.9745699923344944 ) ) ;
#24405=CARTESIAN_POINT ( 'NONE',  ( 7.140644628064522159, -280.8438686885869515, -212.4152043230975835 ) ) ;
#24406=CARTESIAN_POINT ( 'NONE',  ( -5.191159919539834355, -275.2674697424185979, -200.5721390139836160 ) ) ;
#24407=CARTESIAN_POINT ( 'NONE',  ( 3.745638410918268768, -276.6048393869630218, -207.5553387367040727 ) ) ;
#24408=CARTESIAN_POINT ( 'NONE',  ( 22.17056912219155862, -274.7743899400160217, -318.3077515418177086 ) ) ;
#24410=CARTESIAN_POINT ( 'NONE',  ( -37.54014644930101241, -291.2468069710749319, -197.1874386311807257 ) ) ;
#24411=CARTESIAN_POINT ( 'NONE',  ( -106.9169477159257298, -283.4806887771613333, -303.1116555256169818 ) ) ;
#24412=CARTESIAN_POINT ( 'NONE',  ( 24.54194855393093277, -279.2357613747554410, -229.6683071991789689 ) ) ;
#24413=CARTESIAN_POINT ( 'NONE',  ( -2.857032426758452814, -279.0920222158111983, -205.3377278435614244 ) ) ;
#24414=CARTESIAN_POINT ( 'NONE',  ( -42.75491583615490043, -284.0631926679507160, -196.1053225074954014 ) ) ;
#24415=CARTESIAN_POINT ( 'NONE',  ( -90.32403512216293962, -291.8014999248620711, -323.5171117343874130 ) ) ;
#24416=CARTESIAN_POINT ( 'NONE',  ( 0.5920990663355960582, -281.7747204122753715, -207.4679266904495307 ) ) ;
#24417=CARTESIAN_POINT ( 'NONE',  ( -90.47617882071700990, -230.2765427179325286, -347.7368260604238799 ) ) ;
#24418=CARTESIAN_POINT ( 'NONE',  ( 15.18715772473031045, -280.7251099493178685, -325.5622004605534698 ) ) ;
#24419=CARTESIAN_POINT ( 'NONE',  ( 29.14154204925274527, -296.0120784346138407, -305.0739276553849209 ) ) ;
#24420=CARTESIAN_POINT ( 'NONE',  ( -113.2213105307398706, -276.7409103644632182, -274.3933303680112772 ) ) ;
#24421=CARTESIAN_POINT ( 'NONE',  ( -78.14269652366500907, -285.5995863300524888, -333.4904068913745050 ) ) ;
#24422=DIRECTION ( 'NONE',  ( 0.9951408606192336803, 0.000000000000000000, -0.09846150276128748380 ) ) ;
#24423=CARTESIAN_POINT ( 'NONE',  ( -22.50100615812577942, -294.1607292567056220, -196.2195660561077091 ) ) ;
#24424=CARTESIAN_POINT ( 'NONE',  ( 36.34306764750854768, -273.3724385934021370, -256.3769966574627688 ) ) ;
#24426=CARTESIAN_POINT ( 'NONE',  ( -23.80428531193216557, -285.4179281268925479, -194.6704006844306605 ) ) ;
#24427=CARTESIAN_POINT ( 'NONE',  ( -88.47030150166332874, -289.7211053199843604, -217.0710952870387302 ) ) ;
#24429=CARTESIAN_POINT ( 'NONE',  ( 34.37080563932354949, -274.4484211837949488, -286.4980869032250439 ) ) ;
#24430=CARTESIAN_POINT ( 'NONE',  ( -72.73398813780681849, -293.6656382630285975, -335.6309095064376606 ) ) ;
#24431=CARTESIAN_POINT ( 'NONE',  ( -108.8262173792317071, -291.6437048250788280, -287.4259142884952780 ) ) ;
#24434=CARTESIAN_POINT ( 'NONE',  ( 32.77178717436432009, -292.4205988863936341, -300.6077110494586577 ) ) ;
#24435=CARTESIAN_POINT ( 'NONE',  ( 35.35184890735979479, -288.9824010763321667, -257.3419091747679204 ) ) ;
#24436=CARTESIAN_POINT ( 'NONE',  ( -68.95641830046618281, -287.7020170022026946, -339.4729923134647720 ) ) ;
#24437=CARTESIAN_POINT ( 'NONE',  ( -25.06121472957277518, -287.6369597817675867, -197.7520880520980313 ) ) ;
#24440=CARTESIAN_POINT ( 'NONE',  ( 35.71321976717246827, -288.2918730419319218, -265.5659547483629694 ) ) ;
#24441=CARTESIAN_POINT ( 'NONE',  ( 10.18099072548088024, -296.3808755274444593, -328.9091508831531314 ) ) ;
#24443=CARTESIAN_POINT ( 'NONE',  ( 2.521216304964259525, -287.7791631970455342, -204.9473838612087206 ) ) ;
#24444=CARTESIAN_POINT ( 'NONE',  ( -56.58142202532947351, -275.3779631582436309, -343.4846152209454431 ) ) ;
#24446=CARTESIAN_POINT ( 'NONE',  ( -31.44764903199635242, -277.3130646882670476, -347.1666058702533064 ) ) ;
#24448=CARTESIAN_POINT ( 'NONE',  ( -96.79839363741176328, -278.8760408989688813, -221.4463899661410835 ) ) ;
#24449=CARTESIAN_POINT ( 'NONE',  ( -98.23889027957277165, -299.1214885582957663, -227.1942436946234807 ) ) ;
#24450=CARTESIAN_POINT ( 'NONE',  ( -91.07853552446604795, -283.2891324063336924, -217.9668976538289940 ) ) ;
#24452=CARTESIAN_POINT ( 'NONE',  ( -35.61063931487311862, -278.2136496439624125, -196.1334875865333345 ) ) ;
#24453=CARTESIAN_POINT ( 'NONE',  ( -63.24577554830538872, -281.3894433031443327, -340.7456299500937007 ) ) ;
#24455=CARTESIAN_POINT ( 'NONE',  ( 18.38353865410130084, -274.7495234025461741, -322.4898578038768164 ) ) ;
#24457=CARTESIAN_POINT ( 'NONE',  ( -108.5102420067338613, -298.3230722891153164, -251.1879456888849802 ) ) ;
#24458=CARTESIAN_POINT ( 'NONE',  ( -1.789691986299157600, -281.5126062630589558, -338.3136545627217515 ) ) ;
#24459=CARTESIAN_POINT ( 'NONE',  ( -86.26635031143904087, -298.2943618780874999, -215.8653653777751913 ) ) ;
#24460=CARTESIAN_POINT ( 'NONE',  ( -82.69181694050016063, -298.7622603900347258, -208.6781987236896327 ) ) ;
#24461=CARTESIAN_POINT ( 'NONE',  ( -27.28306850219224344, -273.8500880996937212, -197.9851644768884000 ) ) ;
#24462=CARTESIAN_POINT ( 'NONE',  ( 29.25097073197279585, -295.0955987860050413, -235.8587001906870455 ) ) ;
#24463=CARTESIAN_POINT ( 'NONE',  ( 38.97498825534740519, -287.5908240312026010, -260.1257343214477942 ) ) ;
#24464=CARTESIAN_POINT ( 'NONE',  ( -17.34902550193605819, -278.3880463476678528, -197.4940667407226158 ) ) ;
#24465=CARTESIAN_POINT ( 'NONE',  ( -113.1336791305963629, -290.2146312597466249, -284.0214761722375556 ) ) ;
#24466=CARTESIAN_POINT ( 'NONE',  ( -5.701593651523235273, -287.6842543087848298, -336.4089196955332568 ) ) ;
#24467=CARTESIAN_POINT ( 'NONE',  ( -22.56231309923966677, -290.2410455669007661, -196.7788155332748659 ) ) ;
#24469=CARTESIAN_POINT ( 'NONE',  ( 64.33209501061345748, 48.33985520751024723, -319.1928417150128325 ) ) ;
#24470=CARTESIAN_POINT ( 'NONE',  ( 34.81901371492742214, -287.2116075843571252, -281.8784526811728028 ) ) ;
#24472=CARTESIAN_POINT ( 'NONE',  ( -111.2616508970563700, -285.2331650046268692, -291.0652502186668471 ) ) ;
#24474=CARTESIAN_POINT ( 'NONE',  ( 39.42117042560284546, -292.5744765684802928, -267.4574972070860213 ) ) ;
#24475=CARTESIAN_POINT ( 'NONE',  ( -14.39175285408332527, -281.6586652991696837, -197.3220325178714347 ) ) ;
#24476=CARTESIAN_POINT ( 'NONE',  ( -33.49834767716119899, -282.8357820932210416, -343.2724466855644323 ) ) ;
#24477=CARTESIAN_POINT ( 'NONE',  ( -95.57109836026283745, -297.2334133979523472, -219.8996278501121537 ) ) ;
#24478=CARTESIAN_POINT ( 'NONE',  ( 3.188035407583913461, -275.9240371819360007, -208.9930138490575757 ) ) ;
#24479=CARTESIAN_POINT ( 'NONE',  ( 33.36706195070001257, -291.2595873517217910, -246.2810699170521502 ) ) ;
#24480=CARTESIAN_POINT ( 'NONE',  ( -51.62378165303672972, -272.6604384965845043, -198.3149335167148877 ) ) ;
#24483=CARTESIAN_POINT ( 'NONE',  ( 12.07202850344957490, -288.6653354229004549, -214.6178517937098889 ) ) ;
#24484=CARTESIAN_POINT ( 'NONE',  ( -41.91333471279364886, -296.1880208556428329, -346.9678092934881874 ) ) ;
#24485=CARTESIAN_POINT ( 'NONE',  ( -109.2948325731119468, -285.3745483237959206, -257.3817654379772648 ) ) ;
#24486=CARTESIAN_POINT ( 'NONE',  ( 38.50137692911469856, -274.7638586038412427, -282.5539144076752791 ) ) ;
#24487=CARTESIAN_POINT ( 'NONE',  ( 39.50532147334272537, -294.2386464028530781, -273.1625564121264915 ) ) ;
#24488=CARTESIAN_POINT ( 'NONE',  ( 38.40565889229098673, -285.6710715229108928, -268.7353629995159849 ) ) ;
#24489=CARTESIAN_POINT ( 'NONE',  ( -8.392049326693530986, -295.0167837230858368, -341.7454343499975948 ) ) ;
#24490=CARTESIAN_POINT ( 'NONE',  ( -82.55603613438269406, -290.0230144106735111, -327.7000341406693451 ) ) ;
#24491=DIRECTION ( 'NONE',  ( 0.000000000000000000, 0.000000000000000000, -1.000000000000000000 ) ) ;
#24493=CARTESIAN_POINT ( 'NONE',  ( 25.94973956712686558, -24.33012855057486235, -341.4681489864074138 ) ) ;
#24494=CARTESIAN_POINT ( 'NONE',  ( -113.6608146783961644, -286.0409121809512385, -272.8461437193658412 ) ) ;
#24495=CARTESIAN_POINT ( 'NONE',  ( -115.3288506153726871, -276.2666405000204009, -252.5284128619063608 ) ) ;
#24498=CARTESIAN_POINT ( 'NONE',  ( -105.5064114206802657, -283.1114868663364064, -297.4771022698009233 ) ) ;
#24499=CARTESIAN_POINT ( 'NONE',  ( 23.31248646181306938, -284.1506537662010601, -314.2134007783670313 ) ) ;
#24500=CARTESIAN_POINT ( 'NONE',  ( 203.6509206358264521, 291.0907986494672741, -82.86876765886761120 ) ) ;
#24502=CARTESIAN_POINT ( 'NONE',  ( -16.32148925057807531, -281.3604953158954913, -343.8785997295915422 ) ) ;
#24503=CARTESIAN_POINT ( 'NONE',  ( 32.52278763216855140, -285.2275562111103682, -243.9319973170634626 ) ) ;
#24504=CARTESIAN_POINT ( 'NONE',  ( 10.97939469670758150, -276.5726148857862086, -211.9373512105311477 ) ) ;
#24505=CARTESIAN_POINT ( 'NONE',  ( -108.3573470856543395, -296.8175114242272912, -287.5826178669811384 ) ) ;
#24507=CARTESIAN_POINT ( 'NONE',  ( -22.62562070889749322, -290.9293031027489178, -198.3563925603052667 ) ) ;
#24508=CARTESIAN_POINT ( 'NONE',  ( -93.25416783655521158, -278.4810490424109730, -323.2305926496774191 ) ) ;
#24509=CARTESIAN_POINT ( 'NONE',  ( 11.54652308041554853, -274.7527793088335102, -216.0810473614639022 ) ) ;
#24510=CARTESIAN_POINT ( 'NONE',  ( 37.64605842034517025, -274.2698856891760784, -254.2263815589945750 ) ) ;
#24512=CARTESIAN_POINT ( 'NONE',  ( -17.11433242423346712, -272.3129813812006432, -198.0870943656183272 ) ) ;
#24513=CARTESIAN_POINT ( 'NONE',  ( -33.44658098662642232, -296.4293190687830020, -346.6855667789506583 ) ) ;
#24518=CARTESIAN_POINT ( 'NONE',  ( -69.13081775439476928, -284.5600932693857317, -336.4331194644827860 ) ) ;
#24519=CARTESIAN_POINT ( 'NONE',  ( -27.48109341731289135, -284.6887971079321460, -345.7579379232313386 ) ) ;
#24520=CARTESIAN_POINT ( 'NONE',  ( -83.70612531882298413, -284.7450988206101101, -213.7778097407478128 ) ) ;
#24521=CARTESIAN_POINT ( 'NONE',  ( -43.29168214279628302, -275.5284090766885470, -343.9208768822827551 ) ) ;
#24522=CARTESIAN_POINT ( 'NONE',  ( -29.28748367663341057, -284.8095956700114471, -344.2094622355289175 ) ) ;
#24523=CARTESIAN_POINT ( 'NONE',  ( -97.46244542330643412, -276.4423202433099505, -312.9999833993916809 ) ) ;
#24524=CARTESIAN_POINT ( 'NONE',  ( 17.67628227916047834, -277.3208827556949245, -318.8284625850415637 ) ) ;
#24527=CARTESIAN_POINT ( 'NONE',  ( -110.3993511451267153, -279.6570038845173940, -246.3859047144919145 ) ) ;
#24528=CARTESIAN_POINT ( 'NONE',  ( 29.23019569692301900, -281.5424973701628915, -231.7902793948342435 ) ) ;
#24531=CARTESIAN_POINT ( 'NONE',  ( 24.52261197436325091, -288.8240242273793683, -226.5996191902540886 ) ) ;
#24532=CARTESIAN_POINT ( 'NONE',  ( -109.3028118137348201, -295.5746768557292512, -283.6290598565807386 ) ) ;
#24533=CARTESIAN_POINT ( 'NONE',  ( -107.6415570050170203, -289.5010397780856692, -301.6568865569068976 ) ) ;
#24534=CARTESIAN_POINT ( 'NONE',  ( 20.81740448125679777, -285.4969349091684307, -225.2734980637052331 ) ) ;
#24535=CARTESIAN_POINT ( 'NONE',  ( -106.9936658628939483, -288.4632050414346622, -295.3926517285303248 ) ) ;
#24536=CARTESIAN_POINT ( 'NONE',  ( -57.51819236527136070, -286.9910491959993237, -199.7388187287961330 ) ) ;
#24537=CARTESIAN_POINT ( 'NONE',  ( -106.8136892883353255, -276.1835217533882769, -298.6213969685122152 ) ) ;
#24538=CARTESIAN_POINT ( 'NONE',  ( -40.32802213787891787, -287.4889509649636921, -346.5155259750058008 ) ) ;
#24539=CARTESIAN_POINT ( 'NONE',  ( 36.58114696559802326, -289.3887213930033226, -257.6202747898179837 ) ) ;
#24540=CARTESIAN_POINT ( 'NONE',  ( 6.495896134586307546, -284.6456944002850946, -209.2372416867640652 ) ) ;
#24541=CARTESIAN_POINT ( 'NONE',  ( 30.55714785602117445, -282.8597281753982315, -297.8047855580255145 ) ) ;
#24542=CARTESIAN_POINT ( 'NONE',  ( -99.15803628324634644, -291.9737445070194894, -313.1252269025443411 ) ) ;
#24545=CARTESIAN_POINT ( 'NONE',  ( -110.8786663535923083, -298.6936564199741042, -252.9936541290678349 ) ) ;
#24546=CARTESIAN_POINT ( 'NONE',  ( 32.13316527907110043, -280.4436783253834164, -247.2700698265574886 ) ) ;
#24547=CARTESIAN_POINT ( 'NONE',  ( 21.25411053094429903, -278.9083044033890246, -223.5473205831814880 ) ) ;
#24548=CARTESIAN_POINT ( 'NONE',  ( 26.37212219009155589, -293.3164081720143486, -313.3111781230853126 ) ) ;
#24549=CARTESIAN_POINT ( 'NONE',  ( 9.587225927570816708, -297.0490521422769916, -196.5741556780902215 ) ) ;
#24550=CARTESIAN_POINT ( 'NONE',  ( 36.01310505052974520, -280.1779110972923377, -265.8537868321519682 ) ) ;
#24551=CARTESIAN_POINT ( 'NONE',  ( -13.34385970498185259, -274.8180445878520004, -340.8810177047741377 ) ) ;
#24552=CARTESIAN_POINT ( 'NONE',  ( -67.48224483111712857, -296.7711727344507722, -337.4032003638750439 ) ) ;
#24554=CARTESIAN_POINT ( 'NONE',  ( -29.13281317927075875, -296.6330465369202329, -194.0565239425416735 ) ) ;
#24555=CARTESIAN_POINT ( 'NONE',  ( -36.31097824352795556, -293.2792988463515371, -346.3537286391017460 ) ) ;
#24556=CARTESIAN_POINT ( 'NONE',  ( -66.81661364193982422, -293.0834491804830577, -202.9326047874012886 ) ) ;
#24557=CARTESIAN_POINT ( 'NONE',  ( 129.4467878515196162, -299.5541904835127980, -190.0176033293537898 ) ) ;
#24558=CARTESIAN_POINT ( 'NONE',  ( 11.02992459476434028, -293.5446221723825033, -215.4046588239223468 ) ) ;
#24560=CARTESIAN_POINT ( 'NONE',  ( -58.05927619379656335, -281.3384801012228991, -342.8667221965002341 ) ) ;
#24561=CARTESIAN_POINT ( 'NONE',  ( 6.062939907231674752, -294.4449065442651658, -329.1185534946128541 ) ) ;
#24562=CARTESIAN_POINT ( 'NONE',  ( -8.038885970795169200, -282.6789022912734026, -341.6240128786796504 ) ) ;
#24563=CARTESIAN_POINT ( 'NONE',  ( 19.03761677933281504, -282.7770412960509248, -220.0357383591631049 ) ) ;
#24564=CARTESIAN_POINT ( 'NONE',  ( -52.16505365360909963, -285.5342244219547183, -194.7685909183345245 ) ) ;
#24565=CARTESIAN_POINT ( 'NONE',  ( -64.71919363270384906, -289.6937010159547299, -200.7017069746852087 ) ) ;
#24566=CARTESIAN_POINT ( 'NONE',  ( 35.80842208123374348, -280.3090922232262869, -292.2629399496255473 ) ) ;
#24567=CARTESIAN_POINT ( 'NONE',  ( 25.38025973573533278, -285.7127907578231429, -232.0570812730936439 ) ) ;
#24568=CARTESIAN_POINT ( 'NONE',  ( 39.26965611062281880, -286.4158415773543993, -265.8503387409493826 ) ) ;
#24570=CARTESIAN_POINT ( 'NONE',  ( -26.06528609325096468, -296.5063184386654598, -343.2945321364114193 ) ) ;
#24571=CARTESIAN_POINT ( 'NONE',  ( 25.59198146615417713, -277.5549636584964333, -313.7881398116021501 ) ) ;
#24572=CARTESIAN_POINT ( 'NONE',  ( 21.86339244963379613, -292.2095380956092185, -316.9990176015705856 ) ) ;
#24573=CARTESIAN_POINT ( 'NONE',  ( -92.22152547547872814, -278.9063934019443423, -222.1726860815573446 ) ) ;
#24574=CARTESIAN_POINT ( 'NONE',  ( 26.49171239844626058, -293.1503722954759041, -227.2057967811639685 ) ) ;
#24575=CARTESIAN_POINT ( 'NONE',  ( -51.87196184432060875, -283.9476069036426225, -196.1579966918416176 ) ) ;
#24576=CARTESIAN_POINT ( 'NONE',  ( -105.7413767529537125, -280.1474408796800617, -301.2523875054291125 ) ) ;
#24577=CARTESIAN_POINT ( 'NONE',  ( -35.65718105549627381, -294.0892826962033837, -343.5895738469998264 ) ) ;
#24579=CARTESIAN_POINT ( 'NONE',  ( -112.5074205632657680, -270.5881751876177077, -267.5365165288932303 ) ) ;
#24583=CARTESIAN_POINT ( 'NONE',  ( 36.98776750836832150, -283.4366165086683509, -262.9638254481876629 ) ) ;
#24584=CARTESIAN_POINT ( 'NONE',  ( 35.70320008909624931, -293.1011457798167044, -273.4978605523300530 ) ) ;
#24586=CARTESIAN_POINT ( 'NONE',  ( -106.6379572354042296, -276.4809262143061233, -236.9535640164627353 ) ) ;
#24587=CARTESIAN_POINT ( 'NONE',  ( -75.65204922944118948, -296.6130805981129015, -203.7784113293825783 ) ) ;
#24589=CARTESIAN_POINT ( 'NONE',  ( -7.099350016895198401, -289.9787925258967789, -340.6511430220568855 ) ) ;
#24590=CARTESIAN_POINT ( 'NONE',  ( -39.96017090122298754, -288.9191555172766357, -343.3637195597975165 ) ) ;
#24592=CARTESIAN_POINT ( 'NONE',  ( -77.21310500659924969, -281.0275136554026858, -208.3246462274228179 ) ) ;
#24593=CARTESIAN_POINT ( 'NONE',  ( -52.86925619265425524, -299.6107202394247224, -197.9422947700795419 ) ) ;
#24594=CARTESIAN_POINT ( 'NONE',  ( 11.58184918567872934, -279.5441974790371660, -215.6471633970384403 ) ) ;
#24596=CARTESIAN_POINT ( 'NONE',  ( -82.95463243587803959, -297.1140705064888152, -208.2851764265907661 ) ) ;
#24597=CARTESIAN_POINT ( 'NONE',  ( -37.57860526581393401, -293.9693526765320826, -195.9088021524900967 ) ) ;
#24598=CARTESIAN_POINT ( 'NONE',  ( 27.36216727695034123, -294.6190993635756854, -230.0140987193239823 ) ) ;
#24601=CARTESIAN_POINT ( 'NONE',  ( -109.8022962453835589, -291.3357990970879996, -260.3233275407024507 ) ) ;
#24604=CARTESIAN_POINT ( 'NONE',  ( 29.81522044529832982, -291.2305622138032390, -235.1731391212427980 ) ) ;
#24605=CARTESIAN_POINT ( 'NONE',  ( -91.85785198755580439, -296.9133678216314820, -221.7804976360504838 ) ) ;
#24607=CARTESIAN_POINT ( 'NONE',  ( 82.64890176555634582, -299.5541904835127980, -201.5153591320744226 ) ) ;
#24608=CARTESIAN_POINT ( 'NONE',  ( -98.46206618453928172, -291.4586878324099644, -316.0665081189857233 ) ) ;
#24609=CARTESIAN_POINT ( 'NONE',  ( -19.05039376806008633, -291.3376638359844719, -350.3538533559490702 ) ) ;
#24611=CARTESIAN_POINT ( 'NONE',  ( 29.27895320654620903, -289.0992210910067115, -236.1629728259992760 ) ) ;
#24612=CARTESIAN_POINT ( 'NONE',  ( 21.30785965334448306, -272.9118451287024527, -223.8620334824406655 ) ) ;
#24614=CARTESIAN_POINT ( 'NONE',  ( 33.90152715300260411, -277.7530413340703035, -291.9858260242482970 ) ) ;
#24615=CARTESIAN_POINT ( 'NONE',  ( -9.160087433827399650, -290.5032175543380504, -201.4069819873276401 ) ) ;
#24616=CARTESIAN_POINT ( 'NONE',  ( -102.3639107314247951, -280.9290740459282461, -231.3692418883667870 ) ) ;
#24619=CARTESIAN_POINT ( 'NONE',  ( 21.88966573180957909, -281.4995084880939658, -313.2257261522458407 ) ) ;
#24620=CARTESIAN_POINT ( 'NONE',  ( -113.7372913503885172, -279.7235364212798459, -263.0570966039791756 ) ) ;
#24621=CARTESIAN_POINT ( 'NONE',  ( -7.676515842864581884, -279.2273385976901636, -199.7212150923375305 ) ) ;
#24622=CARTESIAN_POINT ( 'NONE',  ( -99.49319086193513328, -245.9241049507712944, -331.6501179397317856 ) ) ;
#24623=CARTESIAN_POINT ( 'NONE',  ( 32.33444253264642754, -276.0784942870038776, -238.0157100554245346 ) ) ;
#24624=PRODUCT_CONTEXT ( 'NONE', #51103, 'mechanical' ) ;
#24625=CARTESIAN_POINT ( 'NONE',  ( -44.00171313750067270, -275.4896595126563170, -194.2928172073101507 ) ) ;
#24626=CARTESIAN_POINT ( 'NONE',  ( -105.5937364680635966, -275.2662352645559167, -254.8156830097664738 ) ) ;
#24629=CARTESIAN_POINT ( 'NONE',  ( -108.9617681973237495, -291.4255923004792521, -286.0652506203121561 ) ) ;
#24630=CARTESIAN_POINT ( 'NONE',  ( -77.58053063487280099, -291.3440424408815943, -334.8803065604809603 ) ) ;
#24631=CARTESIAN_POINT ( 'NONE',  ( -1.199071721370169818, -291.8938201952680629, -206.8044854357036684 ) ) ;
#24632=CARTESIAN_POINT ( 'NONE',  ( -32.30418216715476376, -285.6217007416620390, -193.5745924145047638 ) ) ;
#24634=CARTESIAN_POINT ( 'NONE',  ( -10.70584541269387024, -281.0988842540961627, -339.2409398415281885 ) ) ;
#24635=CARTESIAN_POINT ( 'NONE',  ( 36.86581336776923479, -289.4571033280300867, -273.7937109067386245 ) ) ;
#24636=CARTESIAN_POINT ( 'NONE',  ( -66.85485465257420401, -281.9259172915008094, -337.9002333368860604 ) ) ;
#24637=CARTESIAN_POINT ( 'NONE',  ( -30.23123201532474269, -281.4590228184221701, -197.1620481356565335 ) ) ;
#24638=CARTESIAN_POINT ( 'NONE',  ( 28.70741423731568887, -289.0046157197702996, -309.4806106176583853 ) ) ;
#24639=CARTESIAN_POINT ( 'NONE',  ( -109.3456620402249655, -278.8802702776321212, -282.8212280258921965 ) ) ;
#24640=CARTESIAN_POINT ( 'NONE',  ( -40.60009124559083915, -290.8069889156782892, -193.8144057646714487 ) ) ;
#24641=CARTESIAN_POINT ( 'NONE',  ( -29.48962446833598605, -286.9520443329085992, -193.9248456496801509 ) ) ;
#24642=CARTESIAN_POINT ( 'NONE',  ( 0.2482447686448989166, -287.0312046141614246, -203.2154420724936870 ) ) ;
#24643=CARTESIAN_POINT ( 'NONE',  ( -71.40699958686073501, -283.6819946062201439, -334.9254686515454296 ) ) ;
#24646=CARTESIAN_POINT ( 'NONE',  ( 26.99081124158175271, -294.8793449712281358, -230.2416215306612060 ) ) ;
#24648=CARTESIAN_POINT ( 'NONE',  ( 26.09342928666886507, -292.8041494067347799, -313.1312317169473545 ) ) ;
#24649=CARTESIAN_POINT ( 'NONE',  ( -13.72081148633105485, -275.7967889308401936, -339.7358635659010133 ) ) ;
#24650=CARTESIAN_POINT ( 'NONE',  ( -114.0184817785825402, -295.9820185349875601, -263.8707921404442800 ) ) ;
#24651=CARTESIAN_POINT ( 'NONE',  ( 26.84790489709978090, -291.5399732465593274, -234.0573965944853967 ) ) ;
#24652=CARTESIAN_POINT ( 'NONE',  ( -83.00233680404967629, -293.9262702997888255, -328.6766287563607989 ) ) ;
#24654=CARTESIAN_POINT ( 'NONE',  ( -88.21682213208633527, -292.5258575990554846, -217.3866826588239292 ) ) ;
#24655=CARTESIAN_POINT ( 'NONE',  ( 9.033799285774296806, -293.7854244400997459, -213.5190648787922498 ) ) ;
#24658=CARTESIAN_POINT ( 'NONE',  ( 23.38962777864315967, -292.1544723382924644, -314.6742588820691822 ) ) ;
#24659=CARTESIAN_POINT ( 'NONE',  ( -68.01896229583030618, -299.6495877868003959, -201.9082930060563399 ) ) ;
#24660=CARTESIAN_POINT ( 'NONE',  ( 30.17405039579361414, -288.1123394274220004, -241.8567563461324994 ) ) ;
#24663=CARTESIAN_POINT ( 'NONE',  ( 13.78611618818857920, -278.3199921446559415, -325.7887594672816363 ) ) ;
#24664=CARTESIAN_POINT ( 'NONE',  ( -77.61924689351975815, -276.3746041638488009, -335.5820165320601518 ) ) ;
#24665=CARTESIAN_POINT ( 'NONE',  ( 2.372469025667470977, -273.9182881610584559, -204.5120666990251266 ) ) ;
#24666=CARTESIAN_POINT ( 'NONE',  ( 34.12377414469617776, -279.3617425428742536, -249.5284468617801110 ) ) ;
#24667=CARTESIAN_POINT ( 'NONE',  ( -34.34318743514187844, -275.4149186839528625, -346.5021012867172772 ) ) ;
#24669=CARTESIAN_POINT ( 'NONE',  ( -104.1600173013224406, -295.6483961627992585, -239.6354866054246031 ) ) ;
#24670=CARTESIAN_POINT ( 'NONE',  ( -98.13078375598314551, -275.1513935303307790, -226.3472614259501370 ) ) ;
#24671=CARTESIAN_POINT ( 'NONE',  ( -110.2911103016980974, -273.2753242531903766, -264.9141075488202546 ) ) ;
#24673=CARTESIAN_POINT ( 'NONE',  ( 21.97675669281675681, -286.2072483374698777, -316.8547550167892837 ) ) ;
#24674=CARTESIAN_POINT ( 'NONE',  ( -67.05556151812045584, -273.4848093309479395, -203.6684447092223706 ) ) ;
#24676=CARTESIAN_POINT ( 'NONE',  ( 22.40514260695364612, -288.2040103912519271, -318.9546470363817434 ) ) ;
#24677=CARTESIAN_POINT ( 'NONE',  ( -29.30464945192607118, -300.1321733035788384, -195.0032134068150924 ) ) ;
#24678=CARTESIAN_POINT ( 'NONE',  ( -85.68131689089572944, -293.7223037606157732, -327.5545620920422607 ) ) ;
#24679=CARTESIAN_POINT ( 'NONE',  ( -8.109806667749035469, -281.8761993355265645, -341.4784609991933735 ) ) ;
#24681=CARTESIAN_POINT ( 'NONE',  ( 26.99074920872491035, -279.0346744736479536, -231.7090789594859928 ) ) ;
#24684=CARTESIAN_POINT ( 'NONE',  ( -90.09108366828415626, -290.0806083982209884, -219.3255123637784436 ) ) ;
#24685=CARTESIAN_POINT ( 'NONE',  ( -61.96643003605396416, -281.5151343531188104, -340.4473132351998856 ) ) ;
#24688=CARTESIAN_POINT ( 'NONE',  ( -44.46549000037443733, -289.9619948488783621, -195.6479934131428990 ) ) ;
#24689=CARTESIAN_POINT ( 'NONE',  ( -31.65039828229472008, -284.1869162433017664, -346.7655330158929132 ) ) ;
#24691=CARTESIAN_POINT ( 'NONE',  ( -84.88288915655664368, -271.4821042943038947, -211.6316573950390136 ) ) ;
#24692=CARTESIAN_POINT ( 'NONE',  ( -100.4011321051475960, -284.0474123027393603, -307.1375783713706937 ) ) ;
#24693=CARTESIAN_POINT ( 'NONE',  ( -7.250236046530583067, -278.0747882380499618, -337.5167484837006100 ) ) ;
#24694=CARTESIAN_POINT ( 'NONE',  ( 7.687807447843035824, -277.2224869954009705, -328.0880169124400254 ) ) ;
#24695=CARTESIAN_POINT ( 'NONE',  ( -55.20060866118232923, -285.2820377749279714, -343.2038254532953374 ) ) ;
#24697=CARTESIAN_POINT ( 'NONE',  ( 203.1043581768557544, 295.9636489450775798, -54.00000000006133405 ) ) ;
#24698=CARTESIAN_POINT ( 'NONE',  ( 38.60593156927643577, -293.5451389178173827, -283.1278884188774327 ) ) ;
#24699=CARTESIAN_POINT ( 'NONE',  ( 3.322402274760987595, -288.5815596977761288, -207.7649713208833475 ) ) ;
#24701=CARTESIAN_POINT ( 'NONE',  ( 13.84574458161073807, -284.1952119285919025, -206.2264541496106460 ) ) ;
#24702=CARTESIAN_POINT ( 'NONE',  ( -86.99864850041942077, -276.9200021584703677, -329.0681572795440957 ) ) ;
#24703=CARTESIAN_POINT ( 'NONE',  ( -7.484683838391472221, -290.8369859948538760, -200.2398893648420710 ) ) ;
#24704=CARTESIAN_POINT ( 'NONE',  ( -110.9217803883156819, -286.1366146450784527, -265.4379918796040556 ) ) ;
#24705=CARTESIAN_POINT ( 'NONE',  ( -73.31518544651441971, -279.2962498162957559, -335.0586344776193641 ) ) ;
#24706=CARTESIAN_POINT ( 'NONE',  ( -15.59863551311802610, -287.7532810431171129, -197.0542228195056111 ) ) ;
#24707=CARTESIAN_POINT ( 'NONE',  ( 36.45789534525945186, -283.7248411253985978, -283.7981066141067004 ) ) ;
#24708=CARTESIAN_POINT ( 'NONE',  ( 39.38068138450685751, -275.8005322072798435, -276.8938187662205905 ) ) ;
#24709=CARTESIAN_POINT ( 'NONE',  ( -38.54708760552509261, -276.9001963808065057, -347.3516826353862257 ) ) ;
#24711=CARTESIAN_POINT ( 'NONE',  ( -52.96063129269486325, -299.7707073268676368, -197.5252189089472949 ) ) ;
#24715=CARTESIAN_POINT ( 'NONE',  ( -108.2132656303867861, -271.1454827044902913, -242.8084543558544794 ) ) ;
#24718=CARTESIAN_POINT ( 'NONE',  ( -97.70320141073408138, -277.4875943931880329, -311.5251508827892053 ) ) ;
#24720=CARTESIAN_POINT ( 'NONE',  ( -89.90163341199982483, -274.5351346334454092, -214.5619929788704496 ) ) ;
#24721=CARTESIAN_POINT ( 'NONE',  ( 6.779942849266836546, -281.5271455299173340, -333.2441099510151616 ) ) ;
#24722=CARTESIAN_POINT ( 'NONE',  ( 24.36670301475287914, -288.7519450447548479, -229.4021613922488143 ) ) ;
#24723=CARTESIAN_POINT ( 'NONE',  ( -70.48902961859327831, -297.0012595590896467, -339.1065829002527039 ) ) ;
#24724=CARTESIAN_POINT ( 'NONE',  ( -55.95885352305629823, -296.4918233717499447, -344.6673109744356793 ) ) ;
#24726=CARTESIAN_POINT ( 'NONE',  ( -27.89965840075808856, -294.1723383278712731, -196.0738197769975955 ) ) ;
#24727=CARTESIAN_POINT ( 'NONE',  ( 24.07521869012099103, -280.1333512510219066, -313.1161236590361341 ) ) ;
#24729=CARTESIAN_POINT ( 'NONE',  ( 22.47172739582896028, -282.8627267277936994, -226.0263785211912193 ) ) ;
#24730=CARTESIAN_POINT ( 'NONE',  ( -34.38433971069755302, -296.1692984879676374, -195.9220866594944539 ) ) ;
#24731=CARTESIAN_POINT ( 'NONE',  ( -93.79265034225470288, -285.4494499547828923, -321.5637684949475670 ) ) ;
#24732=CARTESIAN_POINT ( 'NONE',  ( 35.26461582477514156, -286.6066990631442764, -280.5790391357471663 ) ) ;
#24733=CARTESIAN_POINT ( 'NONE',  ( 39.51766203301180269, -280.9312901576506647, -272.8006331946813816 ) ) ;
#24734=CARTESIAN_POINT ( 'NONE',  ( -108.2955140824691966, -267.5841981642410587, -306.8676081293918401 ) ) ;
#24736=CARTESIAN_POINT ( 'NONE',  ( 27.67890005352342442, -286.7661549129841205, -237.0169700876838306 ) ) ;
#24738=CARTESIAN_POINT ( 'NONE',  ( -112.8302213716410733, -285.4583078628263024, -284.1792582437713577 ) ) ;
#24740=CARTESIAN_POINT ( 'NONE',  ( 23.80888718822457761, -275.3325797938629194, -230.4525580281294879 ) ) ;
#24742=CARTESIAN_POINT ( 'NONE',  ( -30.71023853656152625, -291.0543217285215292, -193.9049313277316173 ) ) ;
#24743=CARTESIAN_POINT ( 'NONE',  ( 30.50821717850518411, -282.0270354583017820, -234.3422695862232672 ) ) ;
#24745=CARTESIAN_POINT ( 'NONE',  ( -113.6845556014832113, -280.0923757939359007, -268.7682134599471624 ) ) ;
#24746=CARTESIAN_POINT ( 'NONE',  ( 38.64765668490923645, -282.0403696980138193, -282.7464096631624102 ) ) ;
#24747=CARTESIAN_POINT ( 'NONE',  ( 27.36219212280433055, -278.6237833571632905, -239.2376011013261916 ) ) ;
#24749=CARTESIAN_POINT ( 'NONE',  ( 15.03218479280689834, -278.3119622110595515, -323.8842667980499073 ) ) ;
#24750=CARTESIAN_POINT ( 'NONE',  ( 102.2689123659984034, 116.6942946837412904, -282.5096189404233655 ) ) ;
#24752=CARTESIAN_POINT ( 'NONE',  ( 21.46146779988145070, -280.2061079429810775, -316.3397461528052759 ) ) ;
#24753=CARTESIAN_POINT ( 'NONE',  ( -91.91547213405215189, -296.5952871747879840, -221.7237241646326140 ) ) ;
#24754=CARTESIAN_POINT ( 'NONE',  ( -64.36131451514656021, -291.2166054553856611, -198.2670341956799405 ) ) ;
#24755=CARTESIAN_POINT ( 'NONE',  ( -93.16763214117450786, -239.2410508537212479, -338.7284373407174485 ) ) ;
#24756=CARTESIAN_POINT ( 'NONE',  ( -113.8485494440449344, -271.2371898177336789, -270.3444098319821478 ) ) ;
#24757=CARTESIAN_POINT ( 'NONE',  ( 35.79172722745686031, -285.8180008757970541, -260.0905191214313277 ) ) ;
#24758=CARTESIAN_POINT ( 'NONE',  ( 19.79877908200473158, -296.0734828437670103, -317.7513186455097411 ) ) ;
#24759=CARTESIAN_POINT ( 'NONE',  ( -46.80485354134612663, -287.2448096449472246, -197.4286417822142141 ) ) ;
#24760=CARTESIAN_POINT ( 'NONE',  ( 33.10370670208148169, -294.1035359169013645, -239.8608742318608904 ) ) ;
#24761=CARTESIAN_POINT ( 'NONE',  ( -109.2547132966462300, -285.2155080094811410, -257.3869451307647296 ) ) ;
#24762=CARTESIAN_POINT ( 'NONE',  ( -91.34467392772278060, -296.0992853403963068, -216.0316826934763696 ) ) ;
#24764=CARTESIAN_POINT ( 'NONE',  ( -66.96266101010263583, -292.4764972171892055, -199.4614882434732408 ) ) ;
#24765=CARTESIAN_POINT ( 'NONE',  ( -99.15889336971451939, -291.6541544114275553, -224.5333525818493854 ) ) ;
#24766=CARTESIAN_POINT ( 'NONE',  ( -92.41032733737503690, -290.0348817327506481, -318.3579071300750911 ) ) ;
#24769=CARTESIAN_POINT ( 'NONE',  ( -30.64497133874975887, -299.9955475955708266, -194.5942148631571911 ) ) ;
#24770=CARTESIAN_POINT ( 'NONE',  ( -102.3738020741164974, -271.8794524224558700, -229.8785978720527794 ) ) ;
#24771=CARTESIAN_POINT ( 'NONE',  ( -33.49581723156373414, -282.0613352617378951, -343.5079750332141657 ) ) ;
#24772=ORIENTED_EDGE ( 'NONE', *, *, #68252, .T. ) ;
#24773=CARTESIAN_POINT ( 'NONE',  ( 14.83683626251947629, -275.8481508193265199, -326.9749998273502456 ) ) ;
#24774=CARTESIAN_POINT ( 'NONE',  ( -63.57222284943809854, -272.1043744524579324, -201.3663207359703051 ) ) ;
#24775=CARTESIAN_POINT ( 'NONE',  ( -111.1290831280714997, -280.3010797114725960, -278.9559624860719396 ) ) ;
#24776=CARTESIAN_POINT ( 'NONE',  ( -59.58733595899182234, -275.4829164708435769, -341.1848228058550490 ) ) ;
#24777=CARTESIAN_POINT ( 'NONE',  ( -97.21549071196594127, -298.3467972376506623, -227.9080885675479351 ) ) ;
#24778=CARTESIAN_POINT ( 'NONE',  ( -35.14987133282090781, -299.1598973309951930, -197.0515897046275597 ) ) ;
#24779=CARTESIAN_POINT ( 'NONE',  ( -57.20106889814263695, -299.4003444165638257, -196.7398013132968515 ) ) ;
#24781=CARTESIAN_POINT ( 'NONE',  ( -52.19617784265596327, -271.8831326211135320, -196.4312485482143131 ) ) ;
#24782=CARTESIAN_POINT ( 'NONE',  ( -3.088661111480113242, -295.2383532001938420, -334.9414709280356988 ) ) ;
#24783=CARTESIAN_POINT ( 'NONE',  ( -52.47334284020257655, -290.4293969061633334, -198.2920786537152367 ) ) ;
#24785=CARTESIAN_POINT ( 'NONE',  ( 35.14510787699352790, -276.3720347211612989, -296.3094594296013611 ) ) ;
#24786=CARTESIAN_POINT ( 'NONE',  ( -94.61403151622704399, -273.3575791947326934, -225.0965616287649027 ) ) ;
#24787=CARTESIAN_POINT ( 'NONE',  ( 26.30229587354784115, -280.7994768393588743, -312.8198043207306114 ) ) ;
#24788=CARTESIAN_POINT ( 'NONE',  ( -89.01556573898155023, -282.9983167109281794, -322.2242568858924869 ) ) ;
#24789=CARTESIAN_POINT ( 'NONE',  ( -80.52953097775892388, -281.6355078514125125, -331.9455044203337479 ) ) ;
#24790=CARTESIAN_POINT ( 'NONE',  ( -13.61243191700118338, -275.3128466127583351, -340.0731082936654275 ) ) ;
#24791=CARTESIAN_POINT ( 'NONE',  ( 34.72565397882270588, -283.2828882598632845, -249.4124285421488594 ) ) ;
#24794=CARTESIAN_POINT ( 'NONE',  ( 2.022358464303719572, -272.9697259977997987, -205.1161081648782272 ) ) ;
#24796=CARTESIAN_POINT ( 'NONE',  ( -83.71482780785348154, -279.6866015602371931, -329.5843295770815757 ) ) ;
#24798=CARTESIAN_POINT ( 'NONE',  ( -89.42746297630637287, -285.6986192407990757, -325.1721046157323940 ) ) ;
#24801=CARTESIAN_POINT ( 'NONE',  ( -95.30663867216682661, -289.2084413559330187, -222.7486473314181978 ) ) ;
#24803=CARTESIAN_POINT ( 'NONE',  ( -107.0792717806403687, -295.6510953555426795, -247.3133846204875965 ) ) ;
#24804=CARTESIAN_POINT ( 'NONE',  ( -74.17813100531300563, -287.6867868296533288, -334.8268643047002797 ) ) ;
#24805=CARTESIAN_POINT ( 'NONE',  ( -106.3535322092011199, -272.9508360837029954, -295.9465859460973434 ) ) ;
#24806=CARTESIAN_POINT ( 'NONE',  ( -85.33565360227775898, -295.3892637509222823, -212.6601712253174412 ) ) ;
#24807=CARTESIAN_POINT ( 'NONE',  ( 38.29065932756787305, -285.9042940975855913, -260.2391638466600057 ) ) ;
#24808=CARTESIAN_POINT ( 'NONE',  ( 35.35161745895025120, -282.9861394521215630, -257.6284044288957489 ) ) ;
#24809=CARTESIAN_POINT ( 'NONE',  ( -4.620765952321999492, -280.8668921021031224, -338.9561290907877833 ) ) ;
#24810=CARTESIAN_POINT ( 'NONE',  ( -26.47488923120474169, -288.9101573243335679, -342.5988172604406259 ) ) ;
#24813=CARTESIAN_POINT ( 'NONE',  ( 34.81198186798426519, -283.1675409127749390, -284.8890862866510361 ) ) ;
#24814=CARTESIAN_POINT ( 'NONE',  ( 29.46607840130818801, -282.7571512697327876, -300.3070568979467794 ) ) ;
#24815=CARTESIAN_POINT ( 'NONE',  ( 22.84406396344988721, -290.1489792104142680, -315.7051430209286877 ) ) ;
#24816=CARTESIAN_POINT ( 'NONE',  ( -73.28251617260180240, -297.7559995935917527, -202.2048575721676400 ) ) ;
#24818=CARTESIAN_POINT ( 'NONE',  ( -70.13176940397751480, -273.6320433592557606, -200.6774046727921359 ) ) ;
#24819=CARTESIAN_POINT ( 'NONE',  ( 11.99956529276631656, -294.7214923264852473, -214.2806834480696239 ) ) ;
#24821=CARTESIAN_POINT ( 'NONE',  ( -110.4542110544635705, -280.8376638359844719, -287.0812184334320705 ) ) ;
#24822=CARTESIAN_POINT ( 'NONE',  ( 2.507451714836021139, -274.5195751377456190, -334.1567737173533033 ) ) ;
#24824=CARTESIAN_POINT ( 'NONE',  ( -35.82722352397853172, -296.4706921105976676, -194.1615168451946261 ) ) ;
#24825=CARTESIAN_POINT ( 'NONE',  ( -103.5543086974015949, -291.7154037981345596, -302.9545357144925788 ) ) ;
#24826=CARTESIAN_POINT ( 'NONE',  ( 13.57358983551266363, -274.1371493096339691, -217.9061285539933124 ) ) ;
#24827=CARTESIAN_POINT ( 'NONE',  ( -107.2349525084756863, -292.3795863861720363, -247.0021577344368779 ) ) ;
#24829=CARTESIAN_POINT ( 'NONE',  ( -89.99378689130482201, -292.2265899812234693, -219.4576190109595473 ) ) ;
#24830=CARTESIAN_POINT ( 'NONE',  ( 1.654002269308343376, -284.2835648014221306, -333.3281206238400500 ) ) ;
#24831=CARTESIAN_POINT ( 'NONE',  ( -61.51947899917362150, -293.1695000515571223, -197.8206200288855712 ) ) ;
#24832=CARTESIAN_POINT ( 'NONE',  ( -69.43169095264151736, -292.9538257249130311, -200.8952238960266072 ) ) ;
#24833=CARTESIAN_POINT ( 'NONE',  ( 34.06713222495056925, -293.5862276390502643, -285.5795208352517989 ) ) ;
#24834=CARTESIAN_POINT ( 'NONE',  ( 37.65532829103823076, -289.5608954784788693, -271.0292302036929186 ) ) ;
#24835=CARTESIAN_POINT ( 'NONE',  ( 34.32364353732583595, -281.3601779384821384, -242.0539507915007675 ) ) ;
#24836=CARTESIAN_POINT ( 'NONE',  ( -113.1065001290297971, -270.6920356400427750, -270.3374835933531131 ) ) ;
#24837=CARTESIAN_POINT ( 'NONE',  ( -110.6861932072879000, -284.0902465413399796, -293.8478397423305069 ) ) ;
#24838=CARTESIAN_POINT ( 'NONE',  ( 29.51466977539436698, -277.9736138747033465, -303.6751993177975351 ) ) ;
#24840=CARTESIAN_POINT ( 'NONE',  ( 1.721640143195543038, -284.5744438433160326, -206.3372466918966950 ) ) ;
#24841=CARTESIAN_POINT ( 'NONE',  ( -94.29813285721857596, -276.0046491850214352, -320.3238065899197977 ) ) ;
#24843=CARTESIAN_POINT ( 'NONE',  ( -69.04153268970263468, -282.9883292892177451, -336.2012885968018736 ) ) ;
#24844=CARTESIAN_POINT ( 'NONE',  ( -84.33550593962125674, -280.6271713875945579, -209.7994286087503042 ) ) ;
#24845=CARTESIAN_POINT ( 'NONE',  ( 35.62912769290926462, -286.3081996604329333, -246.3566405324406787 ) ) ;
#24846=CARTESIAN_POINT ( 'NONE',  ( 36.72213116950136680, -295.3172710898968489, -270.7430884814703518 ) ) ;
#24847=CARTESIAN_POINT ( 'NONE',  ( 35.73214306658408645, -277.4266538224841838, -292.0093692451299034 ) ) ;
#24848=CARTESIAN_POINT ( 'NONE',  ( 24.07392711949889730, -276.2567759611323481, -224.7385467734997064 ) ) ;
#24849=CARTESIAN_POINT ( 'NONE',  ( -108.1725979723764510, -278.1517682801263049, -288.0757217756196269 ) ) ;
#24850=CARTESIAN_POINT ( 'NONE',  ( -34.41505128678365111, -300.0890268891578216, -195.5267753367315606 ) ) ;
#24851=CARTESIAN_POINT ( 'NONE',  ( -4.983405806014496342, -284.4789127254735490, -202.8712924513874611 ) ) ;
#24852=CARTESIAN_POINT ( 'NONE',  ( -94.84110387253059571, -291.4692641055593185, -320.3637077735597813 ) ) ;
#24853=CARTESIAN_POINT ( 'NONE',  ( 34.25466151595225028, -292.2647708970275175, -254.5490697432269371 ) ) ;
#24855=CARTESIAN_POINT ( 'NONE',  ( 8.865500545418697698, -292.3726991975644296, -213.7536688816939261 ) ) ;
#24857=CARTESIAN_POINT ( 'NONE',  ( -77.96097736790834176, -290.6636822949068915, -335.4735538706531770 ) ) ;
#24858=CARTESIAN_POINT ( 'NONE',  ( -92.29053374333041404, -279.8909286912926291, -222.1288139876928653 ) ) ;
#24860=CARTESIAN_POINT ( 'NONE',  ( -78.02678613167225308, -296.4391690474578240, -205.3517626077324678 ) ) ;
#24861=CARTESIAN_POINT ( 'NONE',  ( 18.57639655014822821, -288.9253791339152713, -323.1482305238463937 ) ) ;
#24862=CARTESIAN_POINT ( 'NONE',  ( 39.32676735299915549, -287.9718230239024592, -277.2669405668844433 ) ) ;
#24863=CARTESIAN_POINT ( 'NONE',  ( -103.5064205576639580, -285.3038914751115840, -239.3492124669827774 ) ) ;
#24864=CARTESIAN_POINT ( 'NONE',  ( -110.3352075041367044, -266.7738566106981466, -306.9872416995153230 ) ) ;
#24865=CARTESIAN_POINT ( 'NONE',  ( -32.48651102487607290, -123.7208602147541967, -362.7017519726991850 ) ) ;
#24866=CARTESIAN_POINT ( 'NONE',  ( 152.8736219892452084, 204.8876459940559016, -214.3033056176879825 ) ) ;
#24867=EDGE_CURVE ( 'NONE', #8997, #19844, #36751, .T. ) ;
#24868=CARTESIAN_POINT ( 'NONE',  ( 9.760221938220913884, -275.5811667680674191, -326.3433532371472552 ) ) ;
#24869=CARTESIAN_POINT ( 'NONE',  ( -16.30526454057934771, -275.6942111142294038, -340.6403722902391564 ) ) ;
#24870=CARTESIAN_POINT ( 'NONE',  ( -102.6988461933361094, -272.7511064686084410, -229.6894109900751175 ) ) ;
#24871=CARTESIAN_POINT ( 'NONE',  ( 46.35570317780937444, 10.66898867798451711, -328.9001176944748863 ) ) ;
#24872=CARTESIAN_POINT ( 'NONE',  ( -56.81478339010194389, -275.9828458547286800, -344.4029643667979599 ) ) ;
#24874=CARTESIAN_POINT ( 'NONE',  ( -109.7619785483797585, -291.1767587362562608, -260.3268713466939630 ) ) ;
#24875=CARTESIAN_POINT ( 'NONE',  ( -102.1856188433747974, -297.8964342587916008, -229.1370349007989375 ) ) ;
#24876=CARTESIAN_POINT ( 'NONE',  ( -108.3158456690017601, -296.6648648964790027, -300.2007898421544496 ) ) ;
#24877=CARTESIAN_POINT ( 'NONE',  ( -15.59080451184433258, -294.9295197944176721, -340.0985673028386032 ) ) ;
#24880=CARTESIAN_POINT ( 'NONE',  ( -96.78070654838988673, -279.8367358613911051, -317.0121492477230163 ) ) ;
#24881=CARTESIAN_POINT ( 'NONE',  ( 39.46730344522944023, -281.1261653167881036, -275.6629101201901904 ) ) ;
#24882=CARTESIAN_POINT ( 'NONE',  ( -98.25810032709762254, -280.1969703194087629, -229.4859308229065391 ) ) ;
#24883=CARTESIAN_POINT ( 'NONE',  ( -41.30882770459677999, -278.8615603419586364, -346.2571940978824045 ) ) ;
#24884=CARTESIAN_POINT ( 'NONE',  ( -77.82106971138166784, -296.0717852092317912, -208.8442551567145529 ) ) ;
#24886=CARTESIAN_POINT ( 'NONE',  ( -80.81767902855966668, -277.8277672775424207, -329.0027351424697599 ) ) ;
#24887=CARTESIAN_POINT ( 'NONE',  ( -18.59927838776390274, -275.0903058786832958, -195.7885532554267058 ) ) ;
#24889=CARTESIAN_POINT ( 'NONE',  ( -20.62060439594502981, -287.5267595234128635, -345.0726706229452247 ) ) ;
#24890=CARTESIAN_POINT ( 'NONE',  ( -52.17563904481882986, -275.8625448304757697, -196.7896889069208726 ) ) ;
#24891=CARTESIAN_POINT ( 'NONE',  ( 36.66350591572529538, -274.3667745443983677, -289.3830992925116448 ) ) ;
#24893=CARTESIAN_POINT ( 'NONE',  ( -18.44162639572057927, -287.9996593157644611, -341.0918836248139883 ) ) ;
#24894=CARTESIAN_POINT ( 'NONE',  ( -100.9075469566849534, -284.4732473812842386, -226.9924126580549171 ) ) ;
#24895=CARTESIAN_POINT ( 'NONE',  ( 36.43721176719488852, -279.8765894378322514, -276.8621489865867034 ) ) ;
#24896=CARTESIAN_POINT ( 'NONE',  ( 35.06194823852340647, -280.2999618685950622, -283.5878713537687190 ) ) ;
#24897=CARTESIAN_POINT ( 'NONE',  ( -95.22666276784291028, -283.2813603821070387, -223.5365944728001466 ) ) ;
#24898=CARTESIAN_POINT ( 'NONE',  ( -107.9782549589254472, -292.2238796736452855, -295.7218778890996305 ) ) ;
#24899=CARTESIAN_POINT ( 'NONE',  ( -110.6762482752506997, -279.7174939040168056, -273.3900702410109034 ) ) ;
#24901=CARTESIAN_POINT ( 'NONE',  ( 29.05471765238056037, -280.4434695260436570, -307.8578568709908154 ) ) ;
#24902=CARTESIAN_POINT ( 'NONE',  ( 37.50807736187562114, -295.6230021732154114, -275.8662945541850036 ) ) ;
#24903=CARTESIAN_POINT ( 'NONE',  ( -92.32482502241525424, -277.5193871696083647, -217.8376088618541928 ) ) ;
#24904=CARTESIAN_POINT ( 'NONE',  ( -96.96403338409147921, -278.6135046988646877, -312.6802546109517493 ) ) ;
#24905=CARTESIAN_POINT ( 'NONE',  ( -98.28669884495361941, -285.9536657177474126, -314.4450583561402937 ) ) ;
#24907=CARTESIAN_POINT ( 'NONE',  ( -110.2499118893775574, -292.7261145376525064, -250.4699144322435984 ) ) ;
#24908=CARTESIAN_POINT ( 'NONE',  ( 23.92904542599891116, -272.9641282553837982, -227.0850166246396498 ) ) ;
#24909=CARTESIAN_POINT ( 'NONE',  ( 33.71401382126421709, -286.3753444776108950, -240.9775099686389979 ) ) ;
#24910=CARTESIAN_POINT ( 'NONE',  ( -110.4902897636885797, -289.0846206561997747, -260.1989817374006861 ) ) ;
#24912=CARTESIAN_POINT ( 'NONE',  ( -16.25528957513357042, -275.4587464146221691, -340.8176542087514349 ) ) ;
#24913=CARTESIAN_POINT ( 'NONE',  ( -2.586079678399316073, -292.7269300648275134, -335.9577057709979044 ) ) ;
#24916=CARTESIAN_POINT ( 'NONE',  ( -4.881345449857281693, -290.9517714535404025, -201.3029314322459413 ) ) ;
#24917=CARTESIAN_POINT ( 'NONE',  ( -110.7927309066228361, -286.2524253503041791, -262.6868965602805588 ) ) ;
#24918=CARTESIAN_POINT ( 'NONE',  ( 15.95896971949225041, -286.5495437925206943, -324.5915584081482734 ) ) ;
#24920=CARTESIAN_POINT ( 'NONE',  ( -22.35745005580442069, -287.6729373325198367, -198.2612872854854231 ) ) ;
#24922=CARTESIAN_POINT ( 'NONE',  ( 21.30904977161062774, -288.9674995192254414, -314.1164188195903080 ) ) ;
#24923=CARTESIAN_POINT ( 'NONE',  ( 36.98813944515188723, -295.6913644988241572, -282.8282327442788642 ) ) ;
#24925=CARTESIAN_POINT ( 'NONE',  ( 28.35009146148064829, -288.2395190693545715, -230.8558383656643684 ) ) ;
#24926=CARTESIAN_POINT ( 'NONE',  ( -112.7953601776410721, -276.5809232829304847, -274.3685336897104321 ) ) ;
#24927=CARTESIAN_POINT ( 'NONE',  ( -72.82716028268285413, -277.8424262843965380, -338.6877958660033983 ) ) ;
#24928=CARTESIAN_POINT ( 'NONE',  ( 30.89622787397934900, -291.2067725280568879, -237.7910292729779087 ) ) ;
#24929=CARTESIAN_POINT ( 'NONE',  ( -106.3453804656410995, -278.1116579412484953, -304.6496635814437468 ) ) ;
#24930=CARTESIAN_POINT ( 'NONE',  ( -73.66891921500237572, -299.5472930436217780, -205.1523765639574890 ) ) ;
#24932=CARTESIAN_POINT ( 'NONE',  ( -106.4302533154710915, -282.9348318877348447, -241.0425982353069116 ) ) ;
#24934=CARTESIAN_POINT ( 'NONE',  ( -77.03598048211077298, -275.7293076032742647, -333.1529934475112213 ) ) ;
#24935=CARTESIAN_POINT ( 'NONE',  ( 34.68629357844553596, -279.2823340548097804, -249.4112237689645326 ) ) ;
#24937=CARTESIAN_POINT ( 'NONE',  ( -31.52263184620089120, -275.4599605900671122, -346.4977351006015738 ) ) ;
#24938=CARTESIAN_POINT ( 'NONE',  ( -94.46783928043770118, -297.4192576053155221, -316.9353428337039418 ) ) ;
#24939=CARTESIAN_POINT ( 'NONE',  ( -44.40449788088091765, -282.0597083655492838, -346.7792365828987613 ) ) ;
#24940=CARTESIAN_POINT ( 'NONE',  ( -100.1046072116746330, -298.0121672199594514, -232.5235538516555209 ) ) ;
#24941=CARTESIAN_POINT ( 'NONE',  ( -37.62276689743769253, -299.3638691411998707, -193.8547831036573541 ) ) ;
#24942=CARTESIAN_POINT ( 'NONE',  ( 23.07221168254130461, -274.6483834088388107, -229.3234865802773754 ) ) ;
#24943=CARTESIAN_POINT ( 'NONE',  ( 28.93712421303357374, -296.0189989757953981, -305.5737043482777153 ) ) ;
#24944=CARTESIAN_POINT ( 'NONE',  ( 30.36370218936502496, -288.1945058792406371, -307.1465829586874179 ) ) ;
#24945=CARTESIAN_POINT ( 'NONE',  ( -109.9466627088956585, -276.8993537287911977, -249.4366440837386278 ) ) ;
#24947=CARTESIAN_POINT ( 'NONE',  ( -111.6322356973722236, -290.6396176618745812, -250.0647009199813908 ) ) ;
#24949=CARTESIAN_POINT ( 'NONE',  ( 21.35490538856511833, -287.2236969503184127, -314.1784181319326876 ) ) ;
#24950=CARTESIAN_POINT ( 'NONE',  ( -68.76144104770941112, -289.6390286088553694, -202.2457517645097198 ) ) ;
#24953=CARTESIAN_POINT ( 'NONE',  ( -45.37543667678627912, -288.6643358988658861, -342.9796247055635376 ) ) ;
#24955=CARTESIAN_POINT ( 'NONE',  ( -113.2565782013988951, -285.6406976867037315, -258.6193848352294822 ) ) ;
#24957=CARTESIAN_POINT ( 'NONE',  ( -13.92678369418804252, -291.4073269391968211, -197.1988004247917274 ) ) ;
#24958=CARTESIAN_POINT ( 'NONE',  ( 36.20744015962704054, -282.8995747941821151, -250.3877213855793116 ) ) ;
#24959=CARTESIAN_POINT ( 'NONE',  ( 8.239214098517875229, -281.9759987641352836, -208.8487233424524163 ) ) ;
#24960=CARTESIAN_POINT ( 'NONE',  ( -51.01997869538324437, -283.0650301236675546, -342.1197702936550513 ) ) ;
#24961=CARTESIAN_POINT ( 'NONE',  ( -87.46226070252184570, -297.3755750892354968, -211.8363220019750202 ) ) ;
#24962=CARTESIAN_POINT ( 'NONE',  ( -79.14927638261603704, -274.7904860893174259, -209.8561775473375519 ) ) ;
#24963=CARTESIAN_POINT ( 'NONE',  ( -47.18699936406832762, -289.9465539031880326, -196.3684366963796037 ) ) ;
#24965=CARTESIAN_POINT ( 'NONE',  ( -109.9734265859501079, -271.4903272405545067, -259.4424881070290780 ) ) ;
#24968=CARTESIAN_POINT ( 'NONE',  ( -103.5297167917779859, -286.9264217501230974, -236.2955834187858954 ) ) ;
#24969=CARTESIAN_POINT ( 'NONE',  ( -13.86355234574031847, -295.8341141593112411, -343.3698098339721128 ) ) ;
#24970=CARTESIAN_POINT ( 'NONE',  ( -85.79991449087306421, -286.0117269871989834, -215.5605196998682231 ) ) ;
#24972=CARTESIAN_POINT ( 'NONE',  ( -25.81715911984839096, -275.9675261252064615, -346.2558158670120179 ) ) ;
#24973=CARTESIAN_POINT ( 'NONE',  ( 17.41119197392769991, -293.4603246186936758, -216.2913910040802818 ) ) ;
#24974=CARTESIAN_POINT ( 'NONE',  ( 2.118241632445099665, -284.7141658548872556, -205.6833128552913195 ) ) ;
#24975=CARTESIAN_POINT ( 'NONE',  ( -58.93681956333193028, -292.1134500924573558, -196.4733983802848343 ) ) ;
#24976=CARTESIAN_POINT ( 'NONE',  ( -98.12592179381310586, -290.3236088074801273, -310.8482574306502215 ) ) ;
#24979=CARTESIAN_POINT ( 'NONE',  ( -97.49377626717115675, -246.8080880501614160, -331.4215790215362176 ) ) ;
#24980=CARTESIAN_POINT ( 'NONE',  ( -46.44218456700350117, -287.4587736984151434, -194.5990632669329159 ) ) ;
#24981=CARTESIAN_POINT ( 'NONE',  ( -115.3288506153726871, -270.2666405000204009, -252.5284128619063608 ) ) ;
#24983=CARTESIAN_POINT ( 'NONE',  ( -92.80195566311395794, -282.7921144748079314, -318.3217121996497667 ) ) ;
#24984=CARTESIAN_POINT ( 'NONE',  ( -72.83471064475116918, -277.1759716973489276, -338.6838738889823617 ) ) ;
#24985=CARTESIAN_POINT ( 'NONE',  ( -46.71062212207951347, -281.9332393492775282, -196.0641906976348992 ) ) ;
#24986=CARTESIAN_POINT ( 'NONE',  ( -110.7721571745674538, -273.6575316501529187, -283.9782850309709943 ) ) ;
#24987=CARTESIAN_POINT ( 'NONE',  ( -0.6742606778060635797, -281.1496163467268730, -337.4140286614663182 ) ) ;
#24988=CARTESIAN_POINT ( 'NONE',  ( -5.065103836973988471, -284.4991777402587445, -203.0412407449558145 ) ) ;
#24989=CARTESIAN_POINT ( 'NONE',  ( -100.1972861174990470, -274.9799996766089407, -227.9654202172991688 ) ) ;
#24990=CARTESIAN_POINT ( 'NONE',  ( -90.44765811065414596, -296.3216628452820487, -320.6111128458912845 ) ) ;
#24993=CARTESIAN_POINT ( 'NONE',  ( -17.28201242359606837, -291.0012081016744219, -199.6056034263659456 ) ) ;
#24994=CARTESIAN_POINT ( 'NONE',  ( 32.92998674943279269, -276.6026556050021554, -301.5893553594597734 ) ) ;
#24995=CARTESIAN_POINT ( 'NONE',  ( -46.17878014752664484, -273.9369232782852350, -197.8979824119133184 ) ) ;
#24996=CARTESIAN_POINT ( 'NONE',  ( 36.98903739376044086, -274.2352935136458996, -251.4816590320255045 ) ) ;
#24998=CARTESIAN_POINT ( 'NONE',  ( -65.94356194598800869, -271.6777997417465258, -201.0154030631533146 ) ) ;
#25000=CARTESIAN_POINT ( 'NONE',  ( 8.566731766197730025, -295.8621839255966961, -331.4432116953627201 ) ) ;
#25003=CARTESIAN_POINT ( 'NONE',  ( -109.2347950416587423, -285.8201850950070479, -256.0220462485468147 ) ) ;
#25004=CARTESIAN_POINT ( 'NONE',  ( -11.03158101682675962, -284.4741215372958436, -341.7034313487334884 ) ) ;
#25005=CARTESIAN_POINT ( 'NONE',  ( -97.43501274370701992, -284.4801380825769002, -228.7134444345888369 ) ) ;
#25006=CARTESIAN_POINT ( 'NONE',  ( -9.707510823128119526, -275.0849210735937618, -338.8057591944971136 ) ) ;
#25007=CARTESIAN_POINT ( 'NONE',  ( -45.75634227399419984, -285.0202243583240147, -344.1697311921894311 ) ) ;
#25008=CARTESIAN_POINT ( 'NONE',  ( -89.59093267963146445, -276.2846886252912100, -322.4021050304311302 ) ) ;
#25009=CARTESIAN_POINT ( 'NONE',  ( -13.97989637146349828, -275.4421884706039236, -200.8740530103883657 ) ) ;
#25011=CARTESIAN_POINT ( 'NONE',  ( -84.47596062612213075, -280.2249929610514982, -209.6100054281786527 ) ) ;
#25014=CARTESIAN_POINT ( 'NONE',  ( -113.1187155047932009, -286.3811513929716739, -272.8329575074588433 ) ) ;
#25015=CARTESIAN_POINT ( 'NONE',  ( -10.44011714154755843, -293.8890886189444700, -338.3971860635331836 ) ) ;
#25016=CARTESIAN_POINT ( 'NONE',  ( -103.7146442847458871, -289.3934818361951784, -309.2987281090792067 ) ) ;
#25017=CARTESIAN_POINT ( 'NONE',  ( -5.340491729265707477, -284.7188931280256270, -203.6096202944680726 ) ) ;
#25018=CARTESIAN_POINT ( 'NONE',  ( 30.51206343914375196, -285.7461960207598395, -241.7467718533398227 ) ) ;
#25019=CARTESIAN_POINT ( 'NONE',  ( -106.6518019166097133, -289.1353579112077909, -244.2526876159719222 ) ) ;
#25020=CARTESIAN_POINT ( 'NONE',  ( 11.38627293384450567, -287.9503721971141772, -215.4046386658568224 ) ) ;
#25021=CARTESIAN_POINT ( 'NONE',  ( -111.2608893949524429, -276.7148886536036230, -257.6743489519632817 ) ) ;
#25022=CARTESIAN_POINT ( 'NONE',  ( 37.88186166704951319, -286.1097444803992857, -282.8410012723633145 ) ) ;
#25023=CARTESIAN_POINT ( 'NONE',  ( -37.99136011208090480, -288.0441689553572928, -195.3639274009831297 ) ) ;
#25024=CARTESIAN_POINT ( 'NONE',  ( 37.77093731994414583, -285.6031122663101769, -274.3516212825301750 ) ) ;
#25025=CARTESIAN_POINT ( 'NONE',  ( -51.05022569497469220, -284.1727838664469346, -342.3537015419958607 ) ) ;
#25026=CARTESIAN_POINT ( 'NONE',  ( -38.85705544674746648, -291.0712801568224108, -345.5125127034490902 ) ) ;
#25029=CARTESIAN_POINT ( 'NONE',  ( -111.9712159807949661, -298.6240136288494114, -258.4574153217983508 ) ) ;
#25031=CARTESIAN_POINT ( 'NONE',  ( 37.51763268699672693, -279.4930349287114950, -265.7697198595055283 ) ) ;
#25032=CARTESIAN_POINT ( 'NONE',  ( 36.92914289369974767, -292.5016245303645519, -250.6125951860784369 ) ) ;
#25033=CARTESIAN_POINT ( 'NONE',  ( -91.00278830484948855, -294.2295247924969317, -321.0995968437806027 ) ) ;
#25034=CARTESIAN_POINT ( 'NONE',  ( 25.97544773420727537, -280.7472436800305786, -307.7736006643471001 ) ) ;
#25035=CARTESIAN_POINT ( 'NONE',  ( 35.79273305344648293, -273.4524320866204334, -256.4805962555096812 ) ) ;
#25036=CARTESIAN_POINT ( 'NONE',  ( -23.40904018080666660, -296.1856146146727156, -342.5734805678191037 ) ) ;
#25037=CARTESIAN_POINT ( 'NONE',  ( -80.89948854861241045, -272.0486489451860166, -207.5170349825756375 ) ) ;
#25038=CARTESIAN_POINT ( 'NONE',  ( 31.30482865398359493, -292.2165490865659763, -303.0663348960810595 ) ) ;
#25039=CARTESIAN_POINT ( 'NONE',  ( 33.18863640069285736, -294.6996985007515377, -249.1893271684930085 ) ) ;
#25041=CARTESIAN_POINT ( 'NONE',  ( 18.59345203627408694, -293.6864562400584191, -223.2032927594639773 ) ) ;
#25043=CARTESIAN_POINT ( 'NONE',  ( -16.61889146615224178, -280.8059646905417139, -342.8650063351921062 ) ) ;
#25044=CARTESIAN_POINT ( 'NONE',  ( 21.32646748840810247, -294.1612257996205244, -313.8012619570395145 ) ) ;
#25045=CARTESIAN_POINT ( 'NONE',  ( -4.163835559721032809, -282.6267483492400743, -339.8610681934162585 ) ) ;
#25046=CARTESIAN_POINT ( 'NONE',  ( -25.64311122380683372, -282.1202483747762813, -195.7122250675870134 ) ) ;
#25047=CARTESIAN_POINT ( 'NONE',  ( -60.49951579780989164, -285.4266634271404541, -196.8926176604023510 ) ) ;
#25048=CARTESIAN_POINT ( 'NONE',  ( -105.2085444465471937, -288.9671867804702856, -238.8314515452892692 ) ) ;
#25049=CARTESIAN_POINT ( 'NONE',  ( 37.57767975301485563, -279.8492438214120739, -255.8768412473338856 ) ) ;
#25050=CARTESIAN_POINT ( 'NONE',  ( 36.08544527965197801, -286.7519431525928439, -292.5414433792432192 ) ) ;
#25052=CARTESIAN_POINT ( 'NONE',  ( -39.69434706120551226, -296.6822850743748745, -344.1361785667474464 ) ) ;
#25053=CARTESIAN_POINT ( 'NONE',  ( -41.33535911566784193, -278.5267455061195960, -346.6805622605221515 ) ) ;
#25054=CARTESIAN_POINT ( 'NONE',  ( 36.97977237842980003, -291.7322195847041257, -282.8780194435805697 ) ) ;
#25055=CARTESIAN_POINT ( 'NONE',  ( -108.9071200265169779, -278.4110251519225017, -255.7904806030904581 ) ) ;
#25056=CARTESIAN_POINT ( 'NONE',  ( -3.323264629320932251, -292.6556181789358106, -201.2687545031113245 ) ) ;
#25057=CARTESIAN_POINT ( 'NONE',  ( -111.1243629882546742, -282.4243651793003096, -286.6532284566049498 ) ) ;
#25058=CARTESIAN_POINT ( 'NONE',  ( -37.10696594301988682, -279.0493349546974287, -345.3734749490556624 ) ) ;
#25059=CARTESIAN_POINT ( 'NONE',  ( 28.60121606276117490, -293.0420555563247831, -302.3361556639268315 ) ) ;
#25060=CARTESIAN_POINT ( 'NONE',  ( 28.61621260249760113, -296.8776238487828891, -195.3835988277860736 ) ) ;
#25063=CARTESIAN_POINT ( 'NONE',  ( 18.01495856046697952, -293.7385066707562373, -318.0627750461171104 ) ) ;
#25064=PLANE ( 'NONE',  #6668 ) ;
#25065=CARTESIAN_POINT ( 'NONE',  ( 17.36665895637873192, -285.6952119285918457, -314.0302885647153062 ) ) ;
#25066=CARTESIAN_POINT ( 'NONE',  ( -65.44466701188630964, -296.7524811496746224, -198.8687172117747082 ) ) ;
#25067=CARTESIAN_POINT ( 'NONE',  ( -46.46341972090297645, -287.2538587767685385, -194.3999930321851934 ) ) ;
#25068=CARTESIAN_POINT ( 'NONE',  ( 25.69497855006543219, -287.8919922355431709, -307.2764936944447527 ) ) ;
#25069=CARTESIAN_POINT ( 'NONE',  ( -83.42539217835839338, -279.2168902879174084, -327.9333112984667196 ) ) ;
#25070=CARTESIAN_POINT ( 'NONE',  ( -103.4473583112783928, -298.7592330576563882, -236.9600625526651356 ) ) ;
#25071=CARTESIAN_POINT ( 'NONE',  ( -102.5013647381963580, -277.8053727829788500, -236.4666975723167468 ) ) ;
#25073=CARTESIAN_POINT ( 'NONE',  ( -48.96260573817354356, -297.5748347812544807, -194.2108251305076294 ) ) ;
#25074=CARTESIAN_POINT ( 'NONE',  ( -108.3830566885144009, -292.7618007427822135, -248.0821281254899873 ) ) ;
#25075=CARTESIAN_POINT ( 'NONE',  ( 22.55561096220015216, -295.7889791258217542, -317.4856954286067321 ) ) ;
#25077=CARTESIAN_POINT ( 'NONE',  ( -110.4388797586241253, -291.1925874554362963, -271.1947833155672356 ) ) ;
#25079=CARTESIAN_POINT ( 'NONE',  ( 22.15310391925788380, -291.0538936007217785, -223.4290380428915910 ) ) ;
#25080=CARTESIAN_POINT ( 'NONE',  ( -103.8336813317700233, -297.3914678223946453, -231.4673927706366499 ) ) ;
#25081=CARTESIAN_POINT ( 'NONE',  ( -101.2310140975651791, -296.7019934227330964, -235.0023418837693043 ) ) ;
#25084=CARTESIAN_POINT ( 'NONE',  ( -89.00769167969961870, -291.2830545843509640, -326.5156642655576889 ) ) ;
#25085=CARTESIAN_POINT ( 'NONE',  ( -111.2586520408596868, -292.6233781216987495, -305.9938812882205070 ) ) ;
#25086=CARTESIAN_POINT ( 'NONE',  ( -109.8638012882397561, -286.3146966435153900, -288.8157454015562280 ) ) ;
#25087=CARTESIAN_POINT ( 'NONE',  ( 33.81277426305639722, -273.2500782434123607, -247.0194919982113220 ) ) ;
#25088=CARTESIAN_POINT ( 'NONE',  ( -2.256129440645577855, -276.4404837920299656, -204.7081140189993107 ) ) ;
#25089=CARTESIAN_POINT ( 'NONE',  ( -47.16067182951224623, -290.0062824044792933, -196.5715388337401919 ) ) ;
#25090=CARTESIAN_POINT ( 'NONE',  ( -64.62774775184927023, -279.2649063883087024, -341.0973042245017268 ) ) ;
#25092=CARTESIAN_POINT ( 'NONE',  ( -26.73617389350672013, -282.2624118907904176, -342.7410132165962864 ) ) ;
#25093=CARTESIAN_POINT ( 'NONE',  ( -80.04261685321067432, -278.6946497979890296, -334.1284465297387669 ) ) ;
#25094=CARTESIAN_POINT ( 'NONE',  ( 14.90180662687149749, -279.5637330310814832, -214.2651621593729772 ) ) ;
#25095=CARTESIAN_POINT ( 'NONE',  ( -95.53025548571402226, -238.2189646283312356, -339.1223768606931799 ) ) ;
#25096=CARTESIAN_POINT ( 'NONE',  ( 34.49732749125324460, -276.1500600901871394, -243.3060939906405906 ) ) ;
#25099=CARTESIAN_POINT ( 'NONE',  ( -41.17746381798538380, -275.5249504634946334, -194.0991289433486315 ) ) ;
#25100=CARTESIAN_POINT ( 'NONE',  ( -67.74223827176244583, -276.1233781216987495, -207.3071070584150277 ) ) ;
#25103=CARTESIAN_POINT ( 'NONE',  ( -45.38275674166889218, -290.2361010911722019, -343.2278969830596793 ) ) ;
#25104=CARTESIAN_POINT ( 'NONE',  ( -23.47456837290901532, -290.6375113347210686, -345.1251422553833663 ) ) ;
#25105=CARTESIAN_POINT ( 'NONE',  ( -104.1442364373609593, -289.5001548687426975, -300.1730902607314420 ) ) ;
#25106=CARTESIAN_POINT ( 'NONE',  ( 25.49846971219115943, -286.4716410379926401, -225.9465103141010047 ) ) ;
#25108=CARTESIAN_POINT ( 'NONE',  ( 35.48980932413891054, -280.1075186424955632, -282.2779819497087033 ) ) ;
#25109=CARTESIAN_POINT ( 'NONE',  ( 36.89054456648177904, -289.4211734303212324, -271.0239339768702393 ) ) ;
#25110=CARTESIAN_POINT ( 'NONE',  ( -32.11567005307058764, -281.4649067403271374, -343.8689159535326212 ) ) ;
#25111=CARTESIAN_POINT ( 'NONE',  ( -94.33349461238223910, -280.5197139791829386, -223.9587598416172796 ) ) ;
#25112=CARTESIAN_POINT ( 'NONE',  ( 39.11914881985140369, -288.4006570871002850, -262.9679640439396167 ) ) ;
#25113=CARTESIAN_POINT ( 'NONE',  ( -66.09969295732130945, -280.1577006354656305, -203.1837393843491384 ) ) ;
#25114=CARTESIAN_POINT ( 'NONE',  ( -111.1634431910774765, -289.0895005352157341, -290.8149433070904024 ) ) ;
#25115=CARTESIAN_POINT ( 'NONE',  ( -85.41984761917466074, -286.2093962739002109, -210.4223946576599928 ) ) ;
#25116=CARTESIAN_POINT ( 'NONE',  ( -85.47929151680671112, -285.8989608587163502, -210.3419610545740852 ) ) ;
#25117=CARTESIAN_POINT ( 'NONE',  ( -108.7196147447171342, -284.5161726657777876, -285.7238559050579170 ) ) ;
#25118=ORIENTED_EDGE ( 'NONE', *, *, #22764, .F. ) ;
#25120=CARTESIAN_POINT ( 'NONE',  ( 12.44863597966686264, -294.5976484457647757, -213.2539563626215795 ) ) ;
#25121=CARTESIAN_POINT ( 'NONE',  ( 31.74787745047207110, -291.8116552382054465, -237.3756766234327529 ) ) ;
#25122=CARTESIAN_POINT ( 'NONE',  ( -19.20178795123518611, -273.3499643337128191, -199.3553518276607974 ) ) ;
#25123=CARTESIAN_POINT ( 'NONE',  ( -22.12583956799603868, -294.2107332157362976, -345.7387696685323135 ) ) ;
#25124=CARTESIAN_POINT ( 'NONE',  ( -30.72563090472262459, -290.6171782834506985, -196.9653730075692977 ) ) ;
#25125=CARTESIAN_POINT ( 'NONE',  ( -85.14950810018693517, -293.9622843865565756, -326.9296437064185170 ) ) ;
#25126=CARTESIAN_POINT ( 'NONE',  ( -32.14440362602869072, -293.3242137605143967, -197.1355980830198860 ) ) ;
#25128=CARTESIAN_POINT ( 'NONE',  ( 0.7925061022009262102, -290.5589297706146681, -205.5265470059704285 ) ) ;
#25129=CARTESIAN_POINT ( 'NONE',  ( 35.47390695503809610, -295.3209147620497106, -252.3394341053670757 ) ) ;
#25130=CARTESIAN_POINT ( 'NONE',  ( -23.72972316758523803, -289.8153276731919732, -342.3721577262268170 ) ) ;
#25131=CARTESIAN_POINT ( 'NONE',  ( -34.33101972808530178, -278.9943606447806701, -345.6561550612795486 ) ) ;
#25132=CARTESIAN_POINT ( 'NONE',  ( -34.32218799048951041, -275.8099074843981384, -346.9045126413045637 ) ) ;
#25133=CARTESIAN_POINT ( 'NONE',  ( -36.88775850084964958, -297.2548719360385689, -193.5226530337290853 ) ) ;
#25134=CARTESIAN_POINT ( 'NONE',  ( -70.35737331132168038, -277.6934137627417840, -203.6290921608441806 ) ) ;
#25135=CARTESIAN_POINT ( 'NONE',  ( -102.9277226285899758, -276.4401961655864852, -309.2578596960130994 ) ) ;
#25136=CARTESIAN_POINT ( 'NONE',  ( -110.2961260465879576, -295.1152369048035098, -279.6516817937797441 ) ) ;
#25138=CARTESIAN_POINT ( 'NONE',  ( -109.9879886971798157, -273.3109204383923725, -262.2119201555834138 ) ) ;
#25140=CARTESIAN_POINT ( 'NONE',  ( -23.63637687900775930, -286.8980798513205741, -344.5124607947947766 ) ) ;
#25141=CARTESIAN_POINT ( 'NONE',  ( 2.931709498142104131, -274.4424217968935977, -209.4151356217638522 ) ) ;
#25142=CARTESIAN_POINT ( 'NONE',  ( 37.82494409277387604, -287.7617935739439758, -287.1238747688250328 ) ) ;
#25143=CARTESIAN_POINT ( 'NONE',  ( -34.85324837914217966, -300.0630427749880482, -195.0050747326455678 ) ) ;
#25144=CARTESIAN_POINT ( 'NONE',  ( -112.2188999222151864, -294.5377763305235703, -271.4653726716557003 ) ) ;
#25146=CARTESIAN_POINT ( 'NONE',  ( -67.82670965532517471, -282.6393887781904937, -340.8935432561564767 ) ) ;
#25149=CARTESIAN_POINT ( 'NONE',  ( -42.99027323350390617, -277.9808197747851182, -195.5229303319318319 ) ) ;
#25151=CARTESIAN_POINT ( 'NONE',  ( -65.46498868004236726, -290.4710229748278039, -202.5521695197263909 ) ) ;
#25154=CARTESIAN_POINT ( 'NONE',  ( -96.68158721091300833, -289.1805867935663628, -224.4941532505116015 ) ) ;
#25155=CARTESIAN_POINT ( 'NONE',  ( -21.80656606556936694, -275.7750136912459880, -198.3238542910373781 ) ) ;
#25156=CARTESIAN_POINT ( 'NONE',  ( 38.08911892454495529, -283.1321845092203375, -282.6412405056415764 ) ) ;
#25157=CARTESIAN_POINT ( 'NONE',  ( 17.90906207888829726, -296.7606155457845034, -195.0244414490978215 ) ) ;
#25158=CARTESIAN_POINT ( 'NONE',  ( -70.21492497528232946, -283.4978458239715451, -335.5544728161844432 ) ) ;
#25159=CARTESIAN_POINT ( 'NONE',  ( 5.505204031250785945, -276.0699991422507651, -210.4690768661828599 ) ) ;
#25160=CARTESIAN_POINT ( 'NONE',  ( -4.040294945074710320, -275.3058196584017310, -205.2039958640114037 ) ) ;
#25161=CARTESIAN_POINT ( 'NONE',  ( -60.58695834865802965, -285.3536961951770081, -341.7221410843583271 ) ) ;
#25164=CARTESIAN_POINT ( 'NONE',  ( 32.22911027982584642, -293.8097538677115494, -303.4839243319868274 ) ) ;
#25165=CARTESIAN_POINT ( 'NONE',  ( -108.9631407931277636, -286.2594202610957836, -291.4356343291743769 ) ) ;
#25166=DIRECTION ( 'NONE',  ( 0.000000000000000000, 0.000000000000000000, 1.000000000000000000 ) ) ;
#25167=CARTESIAN_POINT ( 'NONE',  ( -117.3381139276884966, -270.1608578419545665, -261.3154543817420290 ) ) ;
#25168=CARTESIAN_POINT ( 'NONE',  ( -42.80491282601077785, -276.3166167435363150, -347.0051792499501744 ) ) ;
#25169=CARTESIAN_POINT ( 'NONE',  ( -77.72984708707444668, -287.9843144344482653, -335.0387596558152268 ) ) ;
#25170=CARTESIAN_POINT ( 'NONE',  ( -51.12880872620584682, -284.7515606856853765, -342.8053322172132766 ) ) ;
#25171=CARTESIAN_POINT ( 'NONE',  ( -3.382832845664823562, -278.3574796677457357, -336.1240965390247197 ) ) ;
#25172=CARTESIAN_POINT ( 'NONE',  ( -60.34992273855526435, -287.1849336966969872, -197.4415129900818897 ) ) ;
#25173=CARTESIAN_POINT ( 'NONE',  ( 16.68282718286465283, -282.8204410232708028, -218.2643534992610057 ) ) ;
#25174=CARTESIAN_POINT ( 'NONE',  ( 38.92388368347735650, -275.5861456202410977, -259.7516537931156222 ) ) ;
#25175=CARTESIAN_POINT ( 'NONE',  ( -48.49608528405272523, -277.0235862677593559, -346.6028048552147993 ) ) ;
#25176=CARTESIAN_POINT ( 'NONE',  ( -41.98206177234902725, -299.9133670332113297, -196.0658876998973597 ) ) ;
#25178=CARTESIAN_POINT ( 'NONE',  ( -95.99890600148557951, -281.6948066931273615, -223.6242672951989618 ) ) ;
#25179=CARTESIAN_POINT ( 'NONE',  ( -33.39053363272466157, -296.2407055138936585, -194.5975469267984010 ) ) ;
#25181=CARTESIAN_POINT ( 'NONE',  ( -53.97402699466512388, -276.7790018905211014, -341.5564983688221332 ) ) ;
#25182=CARTESIAN_POINT ( 'NONE',  ( 0.9834008940867228210, -275.7567751832115732, -204.0194830156026455 ) ) ;
#25183=CARTESIAN_POINT ( 'NONE',  ( 36.24966276459002756, -280.8878687597151043, -292.3872257591397670 ) ) ;
#25184=CARTESIAN_POINT ( 'NONE',  ( 32.79378289114194445, -289.0025066346683502, -246.7181901884279682 ) ) ;
#25185=CARTESIAN_POINT ( 'NONE',  ( -112.5173958698081407, -297.9033231660807814, -283.7482983842118074 ) ) ;
#25186=CARTESIAN_POINT ( 'NONE',  ( -37.67178547851752768, -296.2612328933909112, -346.9763469458639520 ) ) ;
#25187=CARTESIAN_POINT ( 'NONE',  ( -30.66822414133165609, -294.1368928966069802, -195.8259373990516110 ) ) ;
#25188=CARTESIAN_POINT ( 'NONE',  ( -92.63468657255643279, -277.2574126706537072, -219.9357862776953141 ) ) ;
#25189=CARTESIAN_POINT ( 'NONE',  ( -21.91948622416577663, -282.1713169440589581, -197.4833172403596961 ) ) ;
#25190=CARTESIAN_POINT ( 'NONE',  ( -69.86503574326503951, -295.7002740160994563, -203.4018255548325271 ) ) ;
#25191=CARTESIAN_POINT ( 'NONE',  ( -96.19763467012533908, -285.7619750118894331, -318.0919214514875648 ) ) ;
#25192=CARTESIAN_POINT ( 'NONE',  ( 18.90774963471604408, -285.8078206768904579, -223.3285211886541504 ) ) ;
#25193=CARTESIAN_POINT ( 'NONE',  ( -93.43388131815913766, -240.9352012794298048, -341.3099153835386801 ) ) ;
#25195=CARTESIAN_POINT ( 'NONE',  ( 35.67628277333682263, -287.2278293432846681, -271.0405734159317603 ) ) ;
#25197=CARTESIAN_POINT ( 'NONE',  ( -37.30055933580196381, -284.1312777191505461, -347.0650093396591274 ) ) ;
#25198=CARTESIAN_POINT ( 'NONE',  ( -1.716021741578490856, -274.8713905094053871, -206.6059306492987275 ) ) ;
#25199=CARTESIAN_POINT ( 'NONE',  ( 37.33600110609494038, -286.1318820393241822, -253.2368117600678943 ) ) ;
#25200=CARTESIAN_POINT ( 'NONE',  ( -99.77139272779301393, -290.0648481671703394, -225.8187113112333009 ) ) ;
#25201=CARTESIAN_POINT ( 'NONE',  ( -5.053894075478392978, -281.4081619655672171, -200.7168950041703397 ) ) ;
#25203=CARTESIAN_POINT ( 'NONE',  ( -104.1955451656680793, -280.5530532153895251, -233.5742839954862973 ) ) ;
#25204=CARTESIAN_POINT ( 'NONE',  ( 38.23312054843977847, -281.7023473310466102, -255.7258601676017804 ) ) ;
#25205=CARTESIAN_POINT ( 'NONE',  ( -105.5937364680635966, -287.8380690714489560, -285.9065529553535612 ) ) ;
#25206=CARTESIAN_POINT ( 'NONE',  ( -62.97513941457921760, -183.2172664956623009, -362.5461488121814000 ) ) ;
#25208=CARTESIAN_POINT ( 'NONE',  ( 30.83474101785412813, -277.9579614473229867, -301.2156362274538992 ) ) ;
#25209=CARTESIAN_POINT ( 'NONE',  ( 202.4138562182569387, 295.8836489450775957, -54.00000000003736034 ) ) ;
#25210=CARTESIAN_POINT ( 'NONE',  ( 35.83831777116904505, -279.7629271663977306, -285.1403556233622112 ) ) ;
#25211=CARTESIAN_POINT ( 'NONE',  ( -8.748272599226140755, -296.4434134283867479, -340.8184974123483357 ) ) ;
#25212=CARTESIAN_POINT ( 'NONE',  ( -105.0594421304473940, -295.5324056855743038, -297.8965512642938052 ) ) ;
#25213=CARTESIAN_POINT ( 'NONE',  ( -33.53613339093320178, -291.6065071166103166, -193.5168301977918475 ) ) ;
#25215=CARTESIAN_POINT ( 'NONE',  ( -112.3070419704224889, -295.3141535650882474, -255.5018913414270969 ) ) ;
#25216=CARTESIAN_POINT ( 'NONE',  ( 24.90226242880337892, -286.4943325827110243, -310.0112067575118431 ) ) ;
#25217=CARTESIAN_POINT ( 'NONE',  ( 31.74363342494571683, -295.7714731510176307, -297.6695450812549097 ) ) ;
#25218=CARTESIAN_POINT ( 'NONE',  ( -10.58593706380056254, -287.7237911593846320, -201.8977204074249130 ) ) ;
#25220=CARTESIAN_POINT ( 'NONE',  ( 37.19060834858754561, -294.2627866692729413, -251.9830003684886890 ) ) ;
#25221=CARTESIAN_POINT ( 'NONE',  ( -99.07968294639007922, -284.5039165993395045, -309.5251142473516666 ) ) ;
#25222=CARTESIAN_POINT ( 'NONE',  ( -104.2635283825039210, -294.8601048830344666, -307.7452902670593744 ) ) ;
#25223=CARTESIAN_POINT ( 'NONE',  ( -110.2808628256932622, -291.6616932123060906, -246.0276771575050248 ) ) ;
#25224=CARTESIAN_POINT ( 'NONE',  ( -47.74128603324633247, -292.4157796233029103, -194.0749874361701757 ) ) ;
#25225=CARTESIAN_POINT ( 'NONE',  ( -78.17265769043761736, -289.7845943366682491, -330.9350521204080451 ) ) ;
#25228=CARTESIAN_POINT ( 'NONE',  ( -48.80684464599588779, -299.7681786728757061, -195.4160152565822273 ) ) ;
#25229=CARTESIAN_POINT ( 'NONE',  ( -103.8769957264625958, -271.8439022749217884, -232.2933646106326364 ) ) ;
#25230=CARTESIAN_POINT ( 'NONE',  ( 33.68671444085101996, -280.3755698939135073, -252.4671301250645001 ) ) ;
#25232=CARTESIAN_POINT ( 'NONE',  ( 38.66779417274447894, -274.9095495595499870, -258.3562667534898765 ) ) ;
#25233=CARTESIAN_POINT ( 'NONE',  ( -109.2728116222713766, -294.8226935133391748, -286.3805734636300713 ) ) ;
#25234=CARTESIAN_POINT ( 'NONE',  ( 3.838665179277843009, -278.3516282875589241, -332.1271522709898250 ) ) ;
#25235=CARTESIAN_POINT ( 'NONE',  ( 8.105489990007118450, -272.8207661384156495, -211.6634315901055174 ) ) ;
#25236=CARTESIAN_POINT ( 'NONE',  ( -109.7521570903174535, -297.5998672125587632, -282.3551259800321986 ) ) ;
#25237=CARTESIAN_POINT ( 'NONE',  ( -92.08483910244299864, -298.3260921711725473, -221.6023771320925277 ) ) ;
#25239=CARTESIAN_POINT ( 'NONE',  ( -107.0495268115293896, -298.5505482323789010, -239.4530033461889786 ) ) ;
#25240=CARTESIAN_POINT ( 'NONE',  ( -112.6969001285957432, -270.5725786104129043, -270.3359661452269620 ) ) ;
#25241=CARTESIAN_POINT ( 'NONE',  ( 28.82726061175138810, -293.7829783668840378, -239.1681964442797153 ) ) ;
#25242=CARTESIAN_POINT ( 'NONE',  ( -55.13741884599251364, -290.3934756011420859, -198.9560249515514840 ) ) ;
#25244=CARTESIAN_POINT ( 'NONE',  ( 32.49456653272469708, -275.6296617277954510, -237.9476973030945999 ) ) ;
#25245=CARTESIAN_POINT ( 'NONE',  ( -89.24366284580175090, -273.4628928124282652, -219.0270525820155854 ) ) ;
#25246=CARTESIAN_POINT ( 'NONE',  ( 35.72999478662111272, -283.2966628321873372, -251.9509520787949839 ) ) ;
#25247=CARTESIAN_POINT ( 'NONE',  ( -71.53347191452294851, -282.1792009550591729, -338.8024871738685420 ) ) ;
#25249=CARTESIAN_POINT ( 'NONE',  ( -110.0344009423584879, -283.6347179900207607, -279.0674441476498941 ) ) ;
#25250=CARTESIAN_POINT ( 'NONE',  ( -110.1067911311129990, -282.3097460872800184, -289.2608214239889435 ) ) ;
#25251=CARTESIAN_POINT ( 'NONE',  ( 35.93912889016937129, -274.2149443663769262, -277.0912750860239271 ) ) ;
#25252=CARTESIAN_POINT ( 'NONE',  ( -59.36924147933729046, -281.7672785440761913, -198.6153887634210946 ) ) ;
#25255=CARTESIAN_POINT ( 'NONE',  ( -92.57807190576829726, -271.6771615585735731, -217.8503338192332990 ) ) ;
#25256=CARTESIAN_POINT ( 'NONE',  ( -81.44940733752194717, -279.6507961020809034, -331.2260388195819587 ) ) ;
#25259=CARTESIAN_POINT ( 'NONE',  ( -111.7150981210542540, -286.2986547208555521, -283.9862470302665542 ) ) ;
#25262=CARTESIAN_POINT ( 'NONE',  ( -29.83112135436138956, -286.9570422825841547, -345.0355507747944444 ) ) ;
#25264=CARTESIAN_POINT ( 'NONE',  ( -110.4963473120028112, -295.2610165182085211, -276.9199384511147741 ) ) ;
#25265=CARTESIAN_POINT ( 'NONE',  ( -97.57447250935021543, -288.0950306985853899, -313.7532671935239819 ) ) ;
#25267=CARTESIAN_POINT ( 'NONE',  ( -98.49924495541347369, -295.1420787038750291, -226.9473487275503487 ) ) ;
#25268=CARTESIAN_POINT ( 'NONE',  ( 13.79671879221067243, -285.2332663998147950, -213.6547990546205540 ) ) ;
#25269=CARTESIAN_POINT ( 'NONE',  ( -7.696587696186280247, -282.0474224700297441, -202.7632188005093496 ) ) ;
#25270=CARTESIAN_POINT ( 'NONE',  ( -87.66741468874603527, -281.9830977621025454, -327.3637777075008444 ) ) ;
#25271=CARTESIAN_POINT ( 'NONE',  ( 7.979943769627845462, -288.4125489688288440, -327.5882845593636716 ) ) ;
#25272=CARTESIAN_POINT ( 'NONE',  ( -46.54802444680345275, -281.3584437868312875, -197.2985173056615906 ) ) ;
#25273=CARTESIAN_POINT ( 'NONE',  ( -22.17088307361434474, -281.0541752502652457, -198.7378679017543277 ) ) ;
#25274=CARTESIAN_POINT ( 'NONE',  ( -2.537498904906047681, -290.5739818968099257, -337.1972936879895428 ) ) ;
#25275=CARTESIAN_POINT ( 'NONE',  ( 99.18384067648280222, -299.8839462645673848, -193.3572539837404349 ) ) ;
#25277=CARTESIAN_POINT ( 'NONE',  ( -106.8432217404455997, -272.9770507113296389, -237.2169104408783369 ) ) ;
#25278=CARTESIAN_POINT ( 'NONE',  ( -30.68484402586279458, -294.1166278728923089, -196.0137369299496299 ) ) ;
#25280=CARTESIAN_POINT ( 'NONE',  ( 31.95455697924148097, -277.6233781216988064, -236.9535640164627637 ) ) ;
#25281=EDGE_LOOP ( 'NONE', ( #48259, #79972, #92607, #11885 ) ) ;
#25282=CARTESIAN_POINT ( 'NONE',  ( 36.92041395726739239, -273.4019796760302938, -258.6518468044378665 ) ) ;
#25284=CARTESIAN_POINT ( 'NONE',  ( -111.8142459796560928, -295.1566365512167067, -254.1670871884807923 ) ) ;
#25285=CARTESIAN_POINT ( 'NONE',  ( -89.30881257830486675, -272.6449314474696166, -218.9479689669707341 ) ) ;
#25286=CARTESIAN_POINT ( 'NONE',  ( -111.0301178524968719, -292.0611564083727103, -271.2124955562864557 ) ) ;
#25287=CARTESIAN_POINT ( 'NONE',  ( 16.57927784217249112, -284.0328252484292193, -321.1352046807982106 ) ) ;
#25288=CARTESIAN_POINT ( 'NONE',  ( -76.88002984230645609, -292.9592470108124189, -204.9141055977990504 ) ) ;
#25289=CARTESIAN_POINT ( 'NONE',  ( -101.2810941020852624, -292.4242238568601238, -228.2534963741508420 ) ) ;
#25290=CARTESIAN_POINT ( 'NONE',  ( 8.226511291301040529, -294.2422458917769177, -327.4571095112128205 ) ) ;
#25291=CARTESIAN_POINT ( 'NONE',  ( 19.26953764472149899, -288.8696336939174216, -221.1659108086443553 ) ) ;
#25292=CARTESIAN_POINT ( 'NONE',  ( 22.52460511167108237, -282.3683730855884164, -318.8073852795956782 ) ) ;
#25293=CARTESIAN_POINT ( 'NONE',  ( -87.66496115127756639, -293.8278495772934207, -326.7951511929214803 ) ) ;
#25294=CARTESIAN_POINT ( 'NONE',  ( 2.092315352667752038, -282.3727358251757096, -336.4970267429923183 ) ) ;
#25295=CARTESIAN_POINT ( 'NONE',  ( 36.46426520696237361, -277.3869757330227799, -259.1161724500052514 ) ) ;
#25296=CARTESIAN_POINT ( 'NONE',  ( 7.450504543161046378, -284.9090924074130839, -326.4764044574609443 ) ) ;
#25297=CARTESIAN_POINT ( 'NONE',  ( -112.0845800623916659, -276.5341076636472053, -282.7630283427802738 ) ) ;
#25299=CARTESIAN_POINT ( 'NONE',  ( -76.16513041315916155, -283.0936099488778268, -332.3138420805906890 ) ) ;
#25300=CARTESIAN_POINT ( 'NONE',  ( -99.93344424428246953, -280.3445826990167120, -226.1991174904782440 ) ) ;
#25301=CARTESIAN_POINT ( 'NONE',  ( 39.40507359593098613, -286.5900875378303567, -268.7019208138915474 ) ) ;
#25302=CARTESIAN_POINT ( 'NONE',  ( -57.95841259011505286, -293.5424550768269114, -199.2235717470466341 ) ) ;
#25303=CARTESIAN_POINT ( 'NONE',  ( 20.22935160620968631, -277.8340848278626254, -320.3009533331063494 ) ) ;
#25304=CARTESIAN_POINT ( 'NONE',  ( 33.25200280530626173, -276.4882719995125626, -240.7315256981000857 ) ) ;
#25305=CARTESIAN_POINT ( 'NONE',  ( -53.95599249986268831, -277.1046166483944830, -341.4974718154298330 ) ) ;
#25306=CARTESIAN_POINT ( 'NONE',  ( -106.9591993256848923, -274.8856171023163029, -243.2879330334971257 ) ) ;
#25307=CARTESIAN_POINT ( 'NONE',  ( -52.43441197048003488, -283.8582324817880931, -197.0655623691760923 ) ) ;
#25308=CARTESIAN_POINT ( 'NONE',  ( 23.09411230421855876, -292.5807809867879996, -222.6613691358707570 ) ) ;
#25309=CARTESIAN_POINT ( 'NONE',  ( -48.72910882811514455, -290.7948378631049309, -345.7588251744553531 ) ) ;
#25310=CARTESIAN_POINT ( 'NONE',  ( -47.02172961108180260, -290.8466296573629961, -197.6939100939247567 ) ) ;
#25311=ORIENTED_EDGE ( 'NONE', *, *, #80735, .F. ) ;
#25312=CARTESIAN_POINT ( 'NONE',  ( -3.565331672669104890, -291.0639237552227883, -201.8064587554073626 ) ) ;
#25313=CARTESIAN_POINT ( 'NONE',  ( -25.40145526563462397, -291.8751199887706775, -198.2713144429138481 ) ) ;
#25315=CARTESIAN_POINT ( 'NONE',  ( -97.90699785994191018, -291.0009720746564881, -317.4072360133181974 ) ) ;
#25316=CARTESIAN_POINT ( 'NONE',  ( -49.16655620748250044, -280.5488808362643454, -198.2219091803277706 ) ) ;
#25317=CARTESIAN_POINT ( 'NONE',  ( -108.5962795115171389, -295.8353016186897548, -241.8586888524557423 ) ) ;
#25318=CARTESIAN_POINT ( 'NONE',  ( -80.88732289647593632, -286.1297315218801032, -206.9163107511304815 ) ) ;
#25319=CARTESIAN_POINT ( 'NONE',  ( 22.97267074852972613, -287.2449544024692045, -222.5078930308498002 ) ) ;
#25320=CARTESIAN_POINT ( 'NONE',  ( -73.80367000584455184, -283.8835602847856308, -333.6849382195065914 ) ) ;
#25321=CARTESIAN_POINT ( 'NONE',  ( -13.31626158342701771, -91.39965012445205161, -359.9159752948824007 ) ) ;
#25322=CARTESIAN_POINT ( 'NONE',  ( 172.3846408709008244, 243.2224064566618438, -178.8072285208067740 ) ) ;
#25323=CARTESIAN_POINT ( 'NONE',  ( 64.22521439624901518, 46.71045597819469464, -315.3326039784200248 ) ) ;
#25324=CARTESIAN_POINT ( 'NONE',  ( -45.93719516178872198, -276.3609526216555423, -343.0666507131855383 ) ) ;
#25325=CARTESIAN_POINT ( 'NONE',  ( -29.69479536131630582, -275.8735244326393854, -343.3214352640654283 ) ) ;
#25326=CARTESIAN_POINT ( 'NONE',  ( -37.24736439065320326, -297.5609611697809100, -193.4219005745662798 ) ) ;
#25327=CARTESIAN_POINT ( 'NONE',  ( -61.61208932556601070, -183.4966681853139221, -359.3482004706497150 ) ) ;
#25328=CARTESIAN_POINT ( 'NONE',  ( -75.10743839796491272, -276.2293225812792343, -336.8971780247672996 ) ) ;
#25329=CARTESIAN_POINT ( 'NONE',  ( -102.9388032797653807, -274.7736880993315935, -235.9718629566357038 ) ) ;
#25331=CARTESIAN_POINT ( 'NONE',  ( -97.39591930593921631, -290.4649665910751537, -311.9941417160450783 ) ) ;
#25332=CARTESIAN_POINT ( 'NONE',  ( 30.60061854741075393, -299.6853369978908859, -193.5135760210463900 ) ) ;
#25333=CARTESIAN_POINT ( 'NONE',  ( -109.7950203624954071, -297.3715044212949579, -244.4759235628065142 ) ) ;
#25334=CARTESIAN_POINT ( 'NONE',  ( -66.05118267075141603, -295.6053306492599972, -337.4786687174667463 ) ) ;
#25336=CARTESIAN_POINT ( 'NONE',  ( -73.38795866116659283, -279.4465274672778605, -336.7835283423722217 ) ) ;
#25337=CARTESIAN_POINT ( 'NONE',  ( -16.16479937763233465, -282.2932702439318291, -344.3830112493215552 ) ) ;
#25338=CARTESIAN_POINT ( 'NONE',  ( -7.400523337463443596, -277.5908462099307599, -337.1962463293898509 ) ) ;
#25339=CARTESIAN_POINT ( 'NONE',  ( 35.52815801109034766, -277.5866408264053007, -291.9467515334152381 ) ) ;
#25340=CARTESIAN_POINT ( 'NONE',  ( -69.49876373618745617, -296.1950756646697869, -204.1697425683345557 ) ) ;
#25342=CARTESIAN_POINT ( 'NONE',  ( -106.4454159008273137, -279.0333888795598796, -246.6755423743570645 ) ) ;
#25343=CARTESIAN_POINT ( 'NONE',  ( -67.48174188482548175, -274.4695436595636693, -199.6805923499918265 ) ) ;
#25344=CARTESIAN_POINT ( 'NONE',  ( 39.11063933135869775, -286.2879884859008826, -274.4136205686718881 ) ) ;
#25345=CARTESIAN_POINT ( 'NONE',  ( -5.974541806667331478, -276.4646038987892211, -202.2354838096020444 ) ) ;
#25347=CARTESIAN_POINT ( 'NONE',  ( -98.98330885496692133, -289.2054505400968765, -309.7681452801497244 ) ) ;
#25348=CARTESIAN_POINT ( 'NONE',  ( -71.01410266429503793, -284.9679966495662029, -201.2273194856097120 ) ) ;
#25350=CARTESIAN_POINT ( 'NONE',  ( 35.06111417893038151, -279.5914541263940123, -254.9446503329105838 ) ) ;
#25351=CARTESIAN_POINT ( 'NONE',  ( 23.05810360897427103, -280.7081466267550809, -312.3996553762333974 ) ) ;
#25352=CARTESIAN_POINT ( 'NONE',  ( -49.63573658191625526, -283.9741464484075664, -196.8908233047757790 ) ) ;
#25353=CARTESIAN_POINT ( 'NONE',  ( -21.56074910916992593, -290.8501246887855700, -343.7346010612021132 ) ) ;
#25354=CARTESIAN_POINT ( 'NONE',  ( -107.6116862006213779, -280.0363335076874591, -249.1653740100405798 ) ) ;
#25356=CARTESIAN_POINT ( 'NONE',  ( 16.67058882306360346, -279.2044453294562345, -216.5366382635107811 ) ) ;
#25357=CARTESIAN_POINT ( 'NONE',  ( -5.477601988872035754, -294.4714841000851493, -202.4664944626865406 ) ) ;
#25358=CARTESIAN_POINT ( 'NONE',  ( -110.7462384188004165, -277.0417893900952890, -250.6704779151933167 ) ) ;
#25359=CARTESIAN_POINT ( 'NONE',  ( -39.15198378159497139, -277.7268825637064538, -343.4406331806724779 ) ) ;
#25360=CARTESIAN_POINT ( 'NONE',  ( -22.07290868366385439, -284.8571383141285764, -343.9606589548379247 ) ) ;
#25362=CARTESIAN_POINT ( 'NONE',  ( -111.5161538510381547, -292.6567330799762772, -255.8899732335158603 ) ) ;
#25363=CARTESIAN_POINT ( 'NONE',  ( 34.70637808644205791, -286.4109706138750084, -243.6546909327920787 ) ) ;
#25364=CARTESIAN_POINT ( 'NONE',  ( -66.86560970675941462, -290.0585375724083974, -202.7240040591368029 ) ) ;
#25366=CARTESIAN_POINT ( 'NONE',  ( -1.242509074817608861, -275.2477632188437724, -334.4350404483913621 ) ) ;
#25367=CARTESIAN_POINT ( 'NONE',  ( 25.45977718219043595, -292.2305885300951900, -310.0409597163760509 ) ) ;
#25369=CARTESIAN_POINT ( 'NONE',  ( -111.3176030456619685, -289.2689422042759588, -251.5929453563863092 ) ) ;
#25370=CARTESIAN_POINT ( 'NONE',  ( -110.6651808524029690, -286.0372916144630722, -279.1738967997951022 ) ) ;
#25371=CARTESIAN_POINT ( 'NONE',  ( -8.636979200828667658, -286.9215176330077952, -340.7315233392874916 ) ) ;
#25373=CARTESIAN_POINT ( 'NONE',  ( 35.54649439789385212, -289.1112386519912434, -280.5864364919723357 ) ) ;
#25375=CARTESIAN_POINT ( 'NONE',  ( 35.81674259387337145, -288.3637602753262854, -271.0274399146314295 ) ) ;
#25376=CARTESIAN_POINT ( 'NONE',  ( 28.15775018440013611, -296.0276461010991511, -307.7255312880222391 ) ) ;
#25377=CARTESIAN_POINT ( 'NONE',  ( -90.33683986780398811, -275.8743505305516805, -324.2937606923914018 ) ) ;
#25378=CARTESIAN_POINT ( 'NONE',  ( -109.7154302119714373, -278.5523456022054916, -296.7427303703722714 ) ) ;
#25379=CARTESIAN_POINT ( 'NONE',  ( -66.43791542598705746, -289.7539504066996869, -200.6278801774358556 ) ) ;
#25380=CARTESIAN_POINT ( 'NONE',  ( -114.0438979584680226, -278.6440389501078130, -263.0139254115716199 ) ) ;
#25381=CARTESIAN_POINT ( 'NONE',  ( -39.23475806822107614, -300.0082013522594480, -195.7276342458387148 ) ) ;
#25383=CARTESIAN_POINT ( 'NONE',  ( -112.3919468259040855, -282.5450820974854196, -270.8988963351653751 ) ) ;
#25385=CARTESIAN_POINT ( 'NONE',  ( -101.8740739154087009, -277.1859463547153837, -233.6672736551553839 ) ) ;
#25386=CARTESIAN_POINT ( 'NONE',  ( 30.23089727730868503, -279.1220303880001552, -237.7001221877023625 ) ) ;
#25388=CARTESIAN_POINT ( 'NONE',  ( 16.45258848134471918, -274.7848160669978483, -324.5540293011601989 ) ) ;
#25389=CARTESIAN_POINT ( 'NONE',  ( -109.4616437019882795, -298.2709844495605580, -255.1536994388734456 ) ) ;
#25390=CARTESIAN_POINT ( 'NONE',  ( 1.924017938745252287, -281.4598917350016904, -336.2374862363736270 ) ) ;
#25391=CARTESIAN_POINT ( 'NONE',  ( -104.1463484580092569, -297.0889874438032621, -300.4941583035100621 ) ) ;
#25392=CARTESIAN_POINT ( 'NONE',  ( -113.8175555806980412, -297.9124606077208455, -266.7752044999442660 ) ) ;
#25393=CARTESIAN_POINT ( 'NONE',  ( -24.58857008613662387, -273.8859802979326332, -198.4106603393156831 ) ) ;
#25394=CARTESIAN_POINT ( 'NONE',  ( 20.88276312212021324, -294.9010370225440738, -223.0659537655007227 ) ) ;
#25395=CARTESIAN_POINT ( 'NONE',  ( 12.07595248769084861, -286.8838986166870200, -211.2416021627170721 ) ) ;
#25396=CARTESIAN_POINT ( 'NONE',  ( 20.76777738762629255, -274.3567082443536833, -318.9779268699946329 ) ) ;
#25397=CARTESIAN_POINT ( 'NONE',  ( -20.49847264130503177, -288.6750686911897787, -345.5510342762020173 ) ) ;
#25398=CARTESIAN_POINT ( 'NONE',  ( 29.02823163649771487, -286.1942101750606753, -239.4024260699484898 ) ) ;
#25400=CARTESIAN_POINT ( 'NONE',  ( -110.6788002138020488, -288.7543947931842467, -254.5948808906440206 ) ) ;
#25402=CARTESIAN_POINT ( 'NONE',  ( 9.093980818847771985, -59.61193948127866094, -357.4272672779520121 ) ) ;
#25403=CARTESIAN_POINT ( 'NONE',  ( -56.08742402907907376, -288.8077049740932125, -341.0294855659019504 ) ) ;
#25405=CARTESIAN_POINT ( 'NONE',  ( -111.9875264138401292, -285.2680066179402729, -288.3281988650538210 ) ) ;
#25406=CARTESIAN_POINT ( 'NONE',  ( -5.972087058750113364, -291.5132298220748908, -200.2842743670373409 ) ) ;
#25407=CARTESIAN_POINT ( 'NONE',  ( 32.43215797779591014, -282.7575677097264020, -239.7335301161027985 ) ) ;
#25408=CARTESIAN_POINT ( 'NONE',  ( 19.74945074723329341, -282.1721589617825998, -219.4110920227378756 ) ) ;
#25409=CARTESIAN_POINT ( 'NONE',  ( -48.33077754406365756, -283.0292425886395904, -342.5292562572490738 ) ) ;
#25410=CARTESIAN_POINT ( 'NONE',  ( -23.94808513997843491, -278.8813625854842826, -344.2083690371267153 ) ) ;
#25411=CARTESIAN_POINT ( 'NONE',  ( -78.20246349483095116, -297.5186664069001949, -205.0970542331542674 ) ) ;
#25412=CARTESIAN_POINT ( 'NONE',  ( -103.6572200806989628, -274.2928604961148835, -238.6831242018080843 ) ) ;
#25413=CARTESIAN_POINT ( 'NONE',  ( -16.95979391574139328, -290.3365969262440558, -198.4990851546085651 ) ) ;
#25415=CARTESIAN_POINT ( 'NONE',  ( -90.47351426350603276, -272.0735781127592077, -219.7053883047262275 ) ) ;
#25418=CARTESIAN_POINT ( 'NONE',  ( -83.67222396746511492, -285.6132797491057431, -328.6921287446546671 ) ) ;
#25419=CARTESIAN_POINT ( 'NONE',  ( 25.46941863734217648, -295.2162608897929204, -314.3869496283570584 ) ) ;
#25420=CARTESIAN_POINT ( 'NONE',  ( -95.04262091548704916, -285.8352853148911095, -225.4576477110521466 ) ) ;
#25421=CARTESIAN_POINT ( 'NONE',  ( 5.729328823447515262, -275.5426119433953431, -333.9040694209037952 ) ) ;
#25422=CARTESIAN_POINT ( 'NONE',  ( -86.45431405527689606, -292.0424002502364829, -211.1204927577868204 ) ) ;
#25423=CARTESIAN_POINT ( 'NONE',  ( -112.5900617009342284, -282.8039838590052568, -261.5299481777547044 ) ) ;
#25424=CARTESIAN_POINT ( 'NONE',  ( -5.899457512176192964, -292.7875569025314917, -200.0821225246380948 ) ) ;
#25425=CARTESIAN_POINT ( 'NONE',  ( -108.1300205867590165, -291.1224743035724032, -252.3909564375660466 ) ) ;
#25428=CARTESIAN_POINT ( 'NONE',  ( -69.56015552319689732, -196.2844319401296218, -356.7998354135015120 ) ) ;
#25429=CARTESIAN_POINT ( 'NONE',  ( -85.09422673512297308, -286.9265702216204090, -210.8430202850986461 ) ) ;
#25430=CARTESIAN_POINT ( 'NONE',  ( -99.86837403722181250, -270.6952119285918457, -220.4570493818173702 ) ) ;
#25432=CARTESIAN_POINT ( 'NONE',  ( 19.92607102360820193, -279.8286444439469847, -224.5940068429489145 ) ) ;
#25433=CARTESIAN_POINT ( 'NONE',  ( -41.38757935571820212, -276.7684760752744637, -347.2467834828916580 ) ) ;
#25434=CARTESIAN_POINT ( 'NONE',  ( -99.53103344926849161, -281.1173109067062228, -228.6455674257470037 ) ) ;
#25435=CARTESIAN_POINT ( 'NONE',  ( 123.3664110013779123, 147.4260113058992658, -261.7119338772159267 ) ) ;
#25436=CARTESIAN_POINT ( 'NONE',  ( -24.64946485751858063, -281.4681075383765005, -345.7640942132951523 ) ) ;
#25437=CARTESIAN_POINT ( 'NONE',  ( -102.4130865246282127, -283.0629160738077417, -233.6825652546871481 ) ) ;
#25438=CARTESIAN_POINT ( 'NONE',  ( -40.42192789263766173, -299.7742003127527823, -194.3854649232285112 ) ) ;
#25439=B_SPLINE_SURFACE_WITH_KNOTS ( 'NONE', 3, 3, ( 
 ( #44293, #38110, #8320, #88774, #36733, #1679, #58987, #87835, #37202, #23922, #16819, #22986, #767, #79828, #67020, #29652, #51860, #88310, #45677, #50945, #58532, #25321, #46156, #3548, #38592, #54201, #68418, #11580, #54658, #39496, #69346, #10637, #40428, #67495, #18691, #82613, #9711, #82144, #2626, #47073 ),
 ( #47554, #26256, #3077, #39041, #18223, #53747, #83069, #31505, #19160, #32437, #33353, #60393, #89231, #24383, #4476, #83532, #53262, #17300, #75515, #11108, #61336, #39975, #89698, #90173, #91085, #75060, #46614, #10171, #67952, #74584, #4020, #75980, #31961, #60855, #68890, #62250, #24864, #17760, #32895, #61783 ),
 ( #90615, #25776, #76459, #55150, #84012, #6361, #35711, #20090, #33837, #12525, #49897, #34307, #40897, #63213, #5899, #77387, #27675, #78792, #13935, #28150, #41375, #92992, #57039, #62746, #85877, #71234, #21029, #5440, #48971, #35234, #69815, #42794, #64159, #4951, #92045, #70309, #91578, #64625, #93451, #27199 ),
 ( #71710, #55621, #26734, #28606, #84470, #6837, #57495, #19620, #56086, #48488, #86338, #13476, #84938, #56573, #70766, #85426, #48017, #76922, #77867, #13017, #12050, #41853, #34769, #63684, #92507, #20574, #49446, #78334, #42323, #58879, #43721, #79725, #8659, #52220, #57956, #80179, #86811, #50842, #14867, #66899 ),
 ( #36622, #8214, #37991, #43270, #87269, #7284, #21969, #21488, #44649, #1113, #79272, #72619, #44176, #81103, #65544, #7741, #37092, #66001, #659, #9115, #29543, #72168, #80634, #14412, #29994, #58423, #15790, #59341, #22415, #51287, #87725, #15317, #2039, #73083, #73550, #22876, #88193, #51741, #65083, #73998 ),
 ( #30449, #36162, #1566, #37537, #23353, #66448, #16246, #45096, #183, #30929, #59819, #29064, #50368, #53141, #9589, #76338, #11464, #74947, #4359, #16701, #3902, #2511, #45556, #40315, #74456, #39850, #33236, #31388, #10057, #38477, #18103, #54079, #60278, #32316, #17648, #61219, #88660, #23809, #89576, #82021 ),
 ( #89115, #52672, #25659, #82949, #75858, #46956, #17178, #68773, #31847, #90053, #46042, #24266, #38927, #10980, #81553, #69230, #32779, #67381, #61667, #67836, #2961, #60736, #53630, #90499, #82500, #46499, #75402, #25206, #10516, #54541, #39385, #68300, #83409, #47428, #18561, #90963, #26127, #56921, #42195, #55023 ),
 ( #62132, #63092, #26610, #64028, #28032, #83893, #19044, #34188, #34649, #19499, #91920, #47900, #5775, #84350, #55501, #49320, #92869, #4824, #27075, #33707, #6240, #70186, #76802, #69695, #11928, #63561, #49779, #77744, #84815, #35109, #62619, #91459, #85760, #92388, #78675, #55961, #27548, #71584, #48366, #77269 ),
 ( #20910, #71108, #12398, #41244, #19965, #56441, #48838, #85304, #5320, #12895, #13816, #41733, #70647, #20453, #78215, #13354, #42668, #6721, #69593, #62509, #55399, #12297, #91349, #26510, #84251, #19402, #48265, #4723, #77167, #33601, #30436, #29051, #15777, #73070, #59328, #9101, #37080, #87256, #37523, #7729 ),
 ( #22863, #647, #44635, #2025, #30917, #45083, #58410, #16233, #73984, #79713, #37978, #88179, #66886, #22402, #65989, #52207, #57943, #59806, #81089, #86798, #80167, #29530, #14855, #52659, #81539, #51274, #74443, #21956, #88647, #72607, #50829, #16687, #43708, #23795, #9575, #36610, #15305, #65530, #23339, #45542 ),
 ( #87712, #73537, #65072, #171, #1100, #44164, #8201, #29981, #58865, #51728, #80621, #8646, #66433, #1553, #69218, #4347, #18548, #31834, #83398, #47416, #53127, #76326, #61655, #11451, #89564, #10502, #25646, #31375, #40303, #54529, #60264, #53617, #2948, #82007, #26115, #55009, #24734, #47886, #89101, #33224 ),
 ( #83882, #24253, #62120, #76790, #74934, #82487, #17164, #90488, #3890, #10044, #46943, #61206, #75845, #38464, #67368, #39371, #60725, #90951, #19032, #46029, #2497, #68287, #10968, #17635, #3408, #38914, #39836, #46486, #75389, #67823, #32300, #90041, #25193, #54067, #82937, #18089, #68760, #32767, #33694, #78204 ),
 ( #49771, #58645, #34177, #70173, #49310, #84805, #20442, #62605, #51509, #70637, #64500, #91448, #40765, #69683, #6712, #85752, #4813, #55488, #12884, #42184, #41721, #71097, #27063, #92378, #29766, #26598, #77733, #84337, #48354, #11916, #35100, #85292, #19488, #77257, #34639, #42659, #55950, #5308, #27537, #56430 ),
 ( #12387, #41233, #63079, #91909, #5765, #78666, #19955, #63549, #92858, #13343, #48826, #6230, #64018, #28022, #56912, #20899, #13807, #71576, #35586, #93326, #87487, #22637, #16472, #17420, #44414, #88435, #46269, #66219, #80872, #80397, #75173, #45800, #67611, #9831, #73773, #31619, #23584, #24035, #37766, #51983 ),
 ( #45327, #23101, #24500, #52451, #15542, #87949, #8433, #52911, #68068, #2280, #9348, #53382, #1334, #16020, #82267, #81789, #3193, #81325, #74710, #89825, #44871, #8887, #60510, #16938, #10286, #38704, #74229, #66671, #1799, #32077, #2739, #73322, #30684, #89345, #39156, #59584, #60976, #30216, #24986, #38233 ),
 ( #37312, #67146, #31163, #59107, #60049, #88887, #69464, #40549, #11237, #41497, #54313, #75632, #19276, #17877, #4596, #61901, #48134, #91695, #25894, #76104, #26383, #90284, #70427, #90735, #77037, #33469, #26847, #40092, #3674, #12652, #55271, #82725, #84126, #83188, #46729, #61453, #54776, #69934, #83653, #48605 ),
 ( #41011, #10755, #69008, #18335, #68536, #5553, #34423, #4139, #63330, #92161, #62372, #76575, #55735, #39612, #25435, #84587, #12168, #53859, #18817, #5076, #32561, #47191, #33010, #33958, #91215, #19737, #62862, #47674, #11698, #77505, #72731, #43380, #56204, #49555, #50486, #22081, #56690, #72275, #70880, #50951 ),
 ( #34886, #21605, #42438, #93107, #21141, #86928, #28262, #71348, #7394, #64278, #6011, #63797, #92626, #49092, #57150, #79388, #14974, #85991, #13131, #85537, #29179, #13586, #20214, #6479, #78904, #20684, #6947, #58075, #79834, #36275, #78450, #65196, #299, #41967, #43830, #14525, #7852, #35356, #50011, #36739 ),
 ( #35820, #14051, #42914, #71828, #65660, #27318, #64734, #27797, #93561, #85063, #28719, #57604, #77990, #86447, #58538, #29658, #45215, #66116, #23474, #87383, #74117, #88317, #31511, #74590, #59465, #89237, #30567, #60399, #22530, #8778, #24390, #80293, #1229, #774, #53268, #59941, #81677, #23928, #87842, #45683 ),
 ( #58993, #16826, #82151, #37208, #52340, #30111, #38598, #37656, #51402, #8326, #15432, #67026, #22992, #1686, #9718, #81218, #44299, #73207, #9237, #51866, #16364, #80759, #38116, #2162, #17306, #67501, #31051, #46163, #88780, #75066, #15911, #66564, #10177, #44767, #73667, #52798, #39047, #2632, #55156, #91091 ),
 ( #11587, #90179, #32443, #84018, #4957, #10643, #32901, #39503, #12056, #75986, #3083, #75521, #89704, #40434, #55627, #83538, #90621, #40903, #53753, #68424, #69823, #69352, #84476, #39981, #33359, #77394, #61344, #25327, #19166, #4482, #33843, #62257, #61789, #3554, #54207, #19626, #48023, #31968, #83075, #26262 ),
 ( #76928, #17766, #62752, #18229, #67958, #47080, #91584, #11114, #68896, #25783, #26741, #4028, #54665, #48495, #18697, #46620, #47560, #76465, #24871, #12531, #60861, #82619, #13482, #27205, #5905, #43276, #27681, #34313, #56579, #92998, #70772, #21035, #72174, #7290, #21496, #34775, #86345, #50374, #56092, #79278 ),
 ( #78340, #57501, #42329, #36168, #13023, #49903, #64166, #6369, #71240, #65089, #86816, #35240, #77874, #20096, #14419, #6843, #63219, #57962, #35717, #84946, #189, #63690, #92515, #85432, #21974, #29070, #50847, #20580, #49452, #78798, #28156, #13943, #92051, #79730, #57045, #41381, #48978, #70315, #41859, #85883 ),
 ( #42800, #71716, #64631, #93457, #28612, #43726, #37098, #37998, #9597, #44184, #30935, #58429, #38484, #30000, #14872, #22421, #9121, #58885, #80642, #8666, #74464, #15797, #87731, #88666, #51750, #87275, #51293, #80185, #36629, #44656, #66907, #2518, #73557, #665, #73090, #16707, #1119, #7746, #22883, #66455 ),
 ( #45562, #67388, #23815, #8220, #59825, #52678, #29549, #81559, #2046, #31395, #66007, #37544, #60285, #65551, #89122, #24273, #15323, #1572, #30455, #59349, #53148, #72624, #88200, #23359, #52226, #81109, #16252, #45102, #74004, #67843, #33245, #91467, #24755, #3429, #38934, #11472, #47437, #53637, #90507, #10989 ) ),
 .UNSPECIFIED., .F., .F., .F.,
 ( 4, 3, 3, 3, 3, 3, 3, 3, 4 ),
 ( 4, 3, 3, 3, 3, 3, 3, 3, 3, 3, 3, 3, 3, 4 ),
 ( -3.330669073875469621E-15, 0.06249999999999708566, 0.1249999999999975020, 0.1874999999999979183, 0.2499999999999983347, 0.3124999999999987788, 0.3749999999999991673, 0.4374999999999995559, 0.5000000000000000000 ),
 ( -7.331489042931211300E-13, 0.06249999999910264836, 0.1249999999989384464, 0.1874999999987742305, 0.2499999999986100285, 0.3749999999982815968, 0.4999999999979531928, 0.6249999999976247889, 0.6874999999974605869, 0.7499999999972963849, 0.8124999999971321829, 0.8749999999969679809, 0.9374999999968037789, 0.9999999999966395769 ),
 .UNSPECIFIED. ) ;
#25440=CARTESIAN_POINT ( 'NONE',  ( -5.509032888388956550, -295.1140799928280103, -336.1371621343747620 ) ) ;
#25442=CARTESIAN_POINT ( 'NONE',  ( -25.31198342667658707, -290.8933852086360048, -197.8073629383141565 ) ) ;
#25443=CARTESIAN_POINT ( 'NONE',  ( 37.49459235954292069, -276.4257125213072754, -288.1052055941094636 ) ) ;
#25444=CARTESIAN_POINT ( 'NONE',  ( 26.63652656261450247, -275.0707052991883756, -235.1020089541326570 ) ) ;
#25445=CARTESIAN_POINT ( 'NONE',  ( 15.82268886041457812, -273.7045411421397603, -215.0886994298425350 ) ) ;
#25447=CARTESIAN_POINT ( 'NONE',  ( -99.68310566211027890, -271.1166714750369806, -228.5733690296224268 ) ) ;
#25448=CARTESIAN_POINT ( 'NONE',  ( 6.292525700994897164, -295.8980229839523304, -333.1524725929577926 ) ) ;
#25451=CARTESIAN_POINT ( 'NONE',  ( 31.65015953459397124, -282.9623050531744184, -295.2973613425602366 ) ) ;
#25452=CARTESIAN_POINT ( 'NONE',  ( 35.62036314281331784, -283.0420285402008176, -249.0892671829823541 ) ) ;
#25453=CARTESIAN_POINT ( 'NONE',  ( -106.6262642408735388, -284.2118868329184238, -246.8886854162517182 ) ) ;
#25454=CARTESIAN_POINT ( 'NONE',  ( -68.39236274638071222, -275.8668823817476436, -337.3249755719738801 ) ) ;
#25455=CARTESIAN_POINT ( 'NONE',  ( 4.099072374511927741, -284.3480798981710791, -332.0149324341556394 ) ) ;
#25456=CARTESIAN_POINT ( 'NONE',  ( -102.4787064723253849, -276.5669855688445864, -304.8267262778476834 ) ) ;
#25457=CARTESIAN_POINT ( 'NONE',  ( 35.68483565052919460, -276.5400946109438109, -263.3776813487488084 ) ) ;
#25459=CARTESIAN_POINT ( 'NONE',  ( -114.0702159846059942, -279.3034715394155114, -274.4713095234498041 ) ) ;
#25462=CARTESIAN_POINT ( 'NONE',  ( -111.7891118326123205, -286.5947931372634798, -256.0204010818362121 ) ) ;
#25463=CARTESIAN_POINT ( 'NONE',  ( -100.3106522776319878, -295.2374354079971681, -307.7102269042525222 ) ) ;
#25464=CARTESIAN_POINT ( 'NONE',  ( -110.3315174758904078, -290.2076818926813075, -245.9912452338584501 ) ) ;
#25466=CARTESIAN_POINT ( 'NONE',  ( 34.99103750803095636, -285.5879606625928204, -254.6783541169293414 ) ) ;
#25467=CARTESIAN_POINT ( 'NONE',  ( -38.61706088930186809, -284.6106107942260337, -196.7703566605917729 ) ) ;
#25468=CARTESIAN_POINT ( 'NONE',  ( -111.3505679452838137, -288.7814211044070021, -271.1744416007073823 ) ) ;
#25470=CARTESIAN_POINT ( 'NONE',  ( -108.7554054368453080, -285.9802409594319101, -253.3595753269164561 ) ) ;
#25471=CARTESIAN_POINT ( 'NONE',  ( -31.62870805527227702, -274.9799995327869624, -345.1944739464025247 ) ) ;
#25472=CARTESIAN_POINT ( 'NONE',  ( 37.50822985570060553, -285.7715584961492823, -256.0807678992746901 ) ) ;
#25473=CARTESIAN_POINT ( 'NONE',  ( -26.92476022374850686, -288.1846429863961134, -196.0359461834780461 ) ) ;
#25474=CARTESIAN_POINT ( 'NONE',  ( 11.21173076402869562, -286.3811501699633482, -327.7422365859876550 ) ) ;
#25475=CARTESIAN_POINT ( 'NONE',  ( -30.25149832316010645, -281.0851610841808110, -197.4193289838501073 ) ) ;
#25476=CARTESIAN_POINT ( 'NONE',  ( -67.29923345947612745, -291.4442404984839072, -339.3000375110531195 ) ) ;
#25479=CARTESIAN_POINT ( 'NONE',  ( -108.9726681848178202, -298.1636975270963035, -294.4093738988105997 ) ) ;
#25480=CARTESIAN_POINT ( 'NONE',  ( -70.60499417502440167, -277.6134202932714743, -203.1267063012960818 ) ) ;
#25481=CARTESIAN_POINT ( 'NONE',  ( -44.87102674738007835, -291.1564412950571068, -193.8395676426056582 ) ) ;
#25482=CARTESIAN_POINT ( 'NONE',  ( -75.60821979140706617, -295.9326490227792874, -207.1978848992800977 ) ) ;
#25483=CARTESIAN_POINT ( 'NONE',  ( 33.59394399054472302, -279.9842275965743283, -251.0937228892536268 ) ) ;
#25484=CARTESIAN_POINT ( 'NONE',  ( -65.08316163842918911, -271.7667198546649843, -201.2696970755833661 ) ) ;
#25485=CARTESIAN_POINT ( 'NONE',  ( 24.85347470641512757, -295.4056666720099429, -309.6103381518848892 ) ) ;
#25486=CARTESIAN_POINT ( 'NONE',  ( -114.2704648735229114, -287.0519495502702512, -270.3937649182068981 ) ) ;
#25487=CARTESIAN_POINT ( 'NONE',  ( -102.2091707222743082, -271.6592913489806733, -229.9777358706982966 ) ) ;
#25488=CARTESIAN_POINT ( 'NONE',  ( 29.99388428293444164, -292.2523819729739785, -305.5732335597014639 ) ) ;
#25490=CARTESIAN_POINT ( 'NONE',  ( 19.79187067718770265, -294.3262418708314954, -223.9609186868267727 ) ) ;
#25491=DIRECTION ( 'NONE',  ( 0.000000000000000000, 0.000000000000000000, -1.000000000000000000 ) ) ;
#25492=CARTESIAN_POINT ( 'NONE',  ( 34.99921143403249602, -294.5031536899988964, -281.6177096995916713 ) ) ;
#25494=CARTESIAN_POINT ( 'NONE',  ( -89.32219838708532222, -281.7992011353934458, -324.9893994723233277 ) ) ;
#25495=CARTESIAN_POINT ( 'NONE',  ( -39.68903769236293044, -295.0824154072274723, -343.3357989888760926 ) ) ;
#25496=CARTESIAN_POINT ( 'NONE',  ( 9.208804488454413573, -282.4323998628255481, -331.6966747171807697 ) ) ;
#25497=CARTESIAN_POINT ( 'NONE',  ( -83.87379996095796741, -283.3380133866291430, -331.7510615724602303 ) ) ;
#25498=CARTESIAN_POINT ( 'NONE',  ( -76.85793325261528253, -287.5825399555865260, -333.9102780500822973 ) ) ;
#25500=CARTESIAN_POINT ( 'NONE',  ( 36.32082713823489684, -279.7798286983633602, -250.3982111275191471 ) ) ;
#25501=CARTESIAN_POINT ( 'NONE',  ( 20.33132837980222618, -287.1593480809937091, -320.9310140225105101 ) ) ;
#25503=CARTESIAN_POINT ( 'NONE',  ( -66.34901754743862057, -297.0385473537887719, -338.2213858319584006 ) ) ;
#25504=CARTESIAN_POINT ( 'NONE',  ( -4.233606403759325509, -278.0495042174313767, -339.2410320296824580 ) ) ;
#25505=CARTESIAN_POINT ( 'NONE',  ( -54.49363932420450141, -279.4925008586195077, -199.3307516649444722 ) ) ;
#25506=CARTESIAN_POINT ( 'NONE',  ( -22.19586651930662669, -292.4075374037363986, -194.8110721692961533 ) ) ;
#25507=CARTESIAN_POINT ( 'NONE',  ( -41.51453533694849085, -281.1840301448403920, -345.8571577947228661 ) ) ;
#25509=CARTESIAN_POINT ( 'NONE',  ( -45.40851032513277374, -279.1543904687937356, -344.9777172841940001 ) ) ;
#25510=CARTESIAN_POINT ( 'NONE',  ( 11.09538014014875529, -291.8008182981295136, -215.3638676092463413 ) ) ;
#25511=CARTESIAN_POINT ( 'NONE',  ( -107.0207933031602607, -294.9149607289440951, -242.4759629644131564 ) ) ;
#25514=CARTESIAN_POINT ( 'NONE',  ( -0.7325421533888573089, -294.0597661249677799, -333.6466836809093479 ) ) ;
#25516=CARTESIAN_POINT ( 'NONE',  ( 27.36219212280433055, -284.6237833571632905, -239.2376011013261916 ) ) ;
#25517=CARTESIAN_POINT ( 'NONE',  ( 7.829102318185203302, -297.6634640464585004, -193.6034160913901303 ) ) ;
#25518=CARTESIAN_POINT ( 'NONE',  ( 37.64531262887317808, -279.8293697398389099, -281.1894788128539062 ) ) ;
#25519=CARTESIAN_POINT ( 'NONE',  ( -80.67278071948570073, -286.7933854495593096, -207.2438859192855602 ) ) ;
#25520=CARTESIAN_POINT ( 'NONE',  ( -80.40921654590333389, -289.4872022119089934, -329.3662731293612183 ) ) ;
#25521=CARTESIAN_POINT ( 'NONE',  ( -56.76444268348722488, -278.8271484498646373, -341.5018364171720577 ) ) ;
#25522=CARTESIAN_POINT ( 'NONE',  ( -111.1424585658010642, -274.1879552814814929, -267.6277344828209266 ) ) ;
#25523=CARTESIAN_POINT ( 'NONE',  ( -43.25429243011743097, -275.9233979841557129, -343.5196564948855666 ) ) ;
#25525=CARTESIAN_POINT ( 'NONE',  ( -85.19995602203759688, -297.0782090278889314, -210.0674065839109517 ) ) ;
#25526=CARTESIAN_POINT ( 'NONE',  ( -110.0643454393489122, -292.2659387964840221, -286.3178005973772429 ) ) ;
#25527=CARTESIAN_POINT ( 'NONE',  ( 18.95257534434676927, -295.8584623611468487, -321.7935722638098923 ) ) ;
#25529=CARTESIAN_POINT ( 'NONE',  ( -101.7290033820603554, -290.7309109456960527, -305.0829804833109051 ) ) ;
#25531=CARTESIAN_POINT ( 'NONE',  ( -44.75226758132235005, -290.0990284552033245, -194.9075265247618063 ) ) ;
#25533=CARTESIAN_POINT ( 'NONE',  ( -36.18904121649769934, -298.3994932829491518, -193.3821985998950197 ) ) ;
#25534=CARTESIAN_POINT ( 'NONE',  ( -110.4053383380896634, -296.2043874184640231, -271.4592006400954460 ) ) ;
#25536=CARTESIAN_POINT ( 'NONE',  ( -77.75265931866277924, -291.1040618683761636, -335.1503460392802367 ) ) ;
#25537=CARTESIAN_POINT ( 'NONE',  ( -72.02372285203398405, -297.9805209788416391, -342.4524372437778652 ) ) ;
#25538=CARTESIAN_POINT ( 'NONE',  ( -105.1573998014192171, -286.9705025672874967, -238.5986683071902235 ) ) ;
#25539=CARTESIAN_POINT ( 'NONE',  ( -54.61048727381081136, -271.8295515885110945, -197.5475381097988645 ) ) ;
#25540=CARTESIAN_POINT ( 'NONE',  ( -92.19996849581345089, -275.1806113581057502, -220.0244057253776759 ) ) ;
#25541=CARTESIAN_POINT ( 'NONE',  ( -55.33725925972116499, -289.8986734863300967, -198.1290333769163112 ) ) ;
#25542=CARTESIAN_POINT ( 'NONE',  ( -112.9973048250349734, -280.3608846345426286, -274.4274377017377446 ) ) ;
#25543=ORIENTED_EDGE ( 'NONE', *, *, #86873, .F. ) ;
#25544=CARTESIAN_POINT ( 'NONE',  ( -3.581672725288374437, -281.9428431318284538, -335.2145838333082111 ) ) ;
#25545=CARTESIAN_POINT ( 'NONE',  ( -96.80595820798417606, -278.9790802324217225, -318.8119841694697811 ) ) ;
#25546=CARTESIAN_POINT ( 'NONE',  ( 34.95804673666359008, -280.0243634471505629, -244.8894512076283831 ) ) ;
#25547=CARTESIAN_POINT ( 'NONE',  ( -99.77846524029713748, -245.9447597285579263, -331.8384115947385453 ) ) ;
#25548=CARTESIAN_POINT ( 'NONE',  ( 25.87993695760413360, -277.0710214728277947, -313.9944411749354458 ) ) ;
#25551=CARTESIAN_POINT ( 'NONE',  ( 9.073143622236854000, -276.1965237946996581, -209.7940474694468946 ) ) ;
#25552=CARTESIAN_POINT ( 'NONE',  ( -6.998514795304313196, -276.9805209788415823, -207.2794874003663779 ) ) ;
#25555=CARTESIAN_POINT ( 'NONE',  ( -110.6459840678237185, -291.6207767266403721, -271.2025624055261801 ) ) ;
#25556=CARTESIAN_POINT ( 'NONE',  ( 36.52472489985140669, -289.5388456816189660, -288.2410043383971470 ) ) ;
#25557=CARTESIAN_POINT ( 'NONE',  ( -104.7939251305819823, -290.2797902223945243, -242.0498235010827841 ) ) ;
#25558=CARTESIAN_POINT ( 'NONE',  ( -36.55975511180312054, -285.5693750356871305, -193.4136011899824723 ) ) ;
#25560=CARTESIAN_POINT ( 'NONE',  ( -21.23322784865867874, -281.2420776797974895, -342.4342333873068469 ) ) ;
#25561=CARTESIAN_POINT ( 'NONE',  ( 28.13085913905408475, -289.8828506476585858, -305.4592933652411944 ) ) ;
#25562=CARTESIAN_POINT ( 'NONE',  ( -34.84223356253615123, -281.5000972172284719, -344.0246092364137667 ) ) ;
#25563=CARTESIAN_POINT ( 'NONE',  ( -93.47765183090484697, -280.5370700635974117, -222.9076060274694555 ) ) ;
#25564=CARTESIAN_POINT ( 'NONE',  ( -56.61036940264855133, -277.7995390838099752, -340.8885253938986466 ) ) ;
#25565=CARTESIAN_POINT ( 'NONE',  ( -112.7451875362350222, -289.1764033355905212, -283.9379867042000001 ) ) ;
#25566=CARTESIAN_POINT ( 'NONE',  ( -108.8818913653904303, -285.7127718562354062, -242.1778256472043154 ) ) ;
#25567=CARTESIAN_POINT ( 'NONE',  ( -57.74565533973548526, -286.2879989769584199, -196.1222160341933431 ) ) ;
#25568=CARTESIAN_POINT ( 'NONE',  ( -32.14358265104954882, -283.1514364725553605, -343.1758114118758840 ) ) ;
#25571=CARTESIAN_POINT ( 'NONE',  ( -107.6433729033232538, -292.0482053882005857, -298.6096627827807879 ) ) ;
#25572=CARTESIAN_POINT ( 'NONE',  ( 3.946974592896316025, -293.1937691885946720, -334.8326730824973652 ) ) ;
#25573=CARTESIAN_POINT ( 'NONE',  ( 35.25532805655532087, -274.4840342527974144, -260.7133230601266973 ) ) ;
#25574=CARTESIAN_POINT ( 'NONE',  ( -39.11381574257350024, -294.4224349072674727, -347.2387635841055271 ) ) ;
#25575=CARTESIAN_POINT ( 'NONE',  ( -37.53249380121460632, -290.5296337344014432, -196.6554668432187896 ) ) ;
#25576=CARTESIAN_POINT ( 'NONE',  ( -80.76719107979832302, -293.8903964171229291, -330.2960889660752741 ) ) ;
#25577=CARTESIAN_POINT ( 'NONE',  ( -110.7654136604953550, -291.7820896920493396, -268.4667398160805760 ) ) ;
#25578=DIRECTION ( 'NONE',  ( 1.000000000000000000, 0.000000000000000000, 0.000000000000000000 ) ) ;
#25579=CARTESIAN_POINT ( 'NONE',  ( 3.175290891185845510, -290.5944646532404363, -206.9874687977882104 ) ) ;
#25580=CARTESIAN_POINT ( 'NONE',  ( 37.69205350818191391, -295.5314410324865548, -268.7352367069600518 ) ) ;
#25581=CARTESIAN_POINT ( 'NONE',  ( 20.55082093029577450, -289.1232809915065332, -315.2352391286513011 ) ) ;
#25582=CARTESIAN_POINT ( 'NONE',  ( -23.22183395170791442, -278.8524837615598813, -344.4346601042021803 ) ) ;
#25583=CARTESIAN_POINT ( 'NONE',  ( -25.84478731655473283, -275.7037448705905263, -346.0963786839527643 ) ) ;
#25584=CARTESIAN_POINT ( 'NONE',  ( -100.6118826841001805, -296.3264313259777509, -226.7370499274407507 ) ) ;
#25585=CARTESIAN_POINT ( 'NONE',  ( -8.362288971461047993, -274.9073398616443455, -338.4789411597768094 ) ) ;
#25586=CARTESIAN_POINT ( 'NONE',  ( -60.15208332618225029, -277.8341531045858801, -199.4477485087159323 ) ) ;
#25587=CARTESIAN_POINT ( 'NONE',  ( 5.395560307258694621, -275.8498380215813199, -210.6270688818391648 ) ) ;
#25588=CARTESIAN_POINT ( 'NONE',  ( -8.209534443423670780, -275.0768568015299138, -340.7865961927353737 ) ) ;
#25590=CARTESIAN_POINT ( 'NONE',  ( -55.34326304613883707, -298.6175498637403507, -199.3964518560269994 ) ) ;
#25591=AXIS2_PLACEMENT_3D ( 'NONE', #89070, #24219, #1989 ) ;
#25593=CARTESIAN_POINT ( 'NONE',  ( -81.90077662346757847, -287.6761211037696171, -331.1303166103268723 ) ) ;
#25594=CARTESIAN_POINT ( 'NONE',  ( -56.85957220997867267, -273.6268068239612035, -199.9660059718328853 ) ) ;
#25595=CARTESIAN_POINT ( 'NONE',  ( -5.626494891228408513, -288.6464334450402021, -340.5262500410424877 ) ) ;
#25596=CARTESIAN_POINT ( 'NONE',  ( -9.574918072416505055, -288.3657980243124257, -342.1577063819490263 ) ) ;
#25597=CARTESIAN_POINT ( 'NONE',  ( -84.67401047114253743, -275.4017879233168742, -211.9686456848743887 ) ) ;
#25598=CARTESIAN_POINT ( 'NONE',  ( -76.64202284590486158, -293.5788096781457170, -334.1044522067512617 ) ) ;
#25599=CARTESIAN_POINT ( 'NONE',  ( -1.202325990908861719, -279.7164282218247990, -202.5517937134897579 ) ) ;
#25600=CARTESIAN_POINT ( 'NONE',  ( 133.0380396672494783, -299.5541904835127980, -195.3611179825600175 ) ) ;
#25601=CARTESIAN_POINT ( 'NONE',  ( -110.5615960594187470, -276.3426869806426680, -286.6625226823388175 ) ) ;
#25603=CARTESIAN_POINT ( 'NONE',  ( -72.80541811414191500, -290.3665778408421261, -206.0431734116716598 ) ) ;
#25606=CARTESIAN_POINT ( 'NONE',  ( -112.3372061547354832, -288.5414404835573805, -271.1825322819155417 ) ) ;
#25607=CARTESIAN_POINT ( 'NONE',  ( 15.93477411641185881, -276.3440126336588492, -219.3723906221099469 ) ) ;
#25608=CARTESIAN_POINT ( 'NONE',  ( 36.97953357970315125, -283.2017377431821501, -288.1641127980598753 ) ) ;
#25609=CARTESIAN_POINT ( 'NONE',  ( -4.285333808817019197, -296.4841077558293705, -195.0169975265855555 ) ) ;
#25610=CARTESIAN_POINT ( 'NONE',  ( -108.4252987394931154, -284.3322923855890849, -287.0326531900352052 ) ) ;
#25611=CARTESIAN_POINT ( 'NONE',  ( -13.89474671823018248, -275.7877336766558187, -200.6071554270697845 ) ) ;
#25612=CARTESIAN_POINT ( 'NONE',  ( 17.39958941581236118, -275.6622237120047885, -221.7474917221501585 ) ) ;
#25614=CARTESIAN_POINT ( 'NONE',  ( 21.84084554167343484, -284.1843652691930515, -316.4516850225342068 ) ) ;
#25615=CARTESIAN_POINT ( 'NONE',  ( -69.61470576497724494, -272.5372755679247803, -204.5380279468873539 ) ) ;
#25618=CARTESIAN_POINT ( 'NONE',  ( 33.41573010253615195, -293.7738229807613379, -300.8665737748893889 ) ) ;
#25619=CARTESIAN_POINT ( 'NONE',  ( -110.8164321505503978, -286.7028126544021234, -257.1243312004908148 ) ) ;
#25621=CARTESIAN_POINT ( 'NONE',  ( -2.602324593224659921, -271.9809262143061233, -198.2974183793908196 ) ) ;
#25622=CARTESIAN_POINT ( 'NONE',  ( -72.77533261791276686, -276.7064962126826231, -338.5565551892367466 ) ) ;
#25623=CARTESIAN_POINT ( 'NONE',  ( -109.1189367289343721, -288.6239593457595447, -296.1002536608158948 ) ) ;
#25624=CARTESIAN_POINT ( 'NONE',  ( -53.82610694498197290, -284.7875690186324391, -342.2396782832729514 ) ) ;
#25625=CARTESIAN_POINT ( 'NONE',  ( -79.18669764713884263, -279.3850730550349226, -331.4724289833314401 ) ) ;
#25626=CARTESIAN_POINT ( 'NONE',  ( -36.58960276809222734, -287.4866838307142984, -193.9411072039653732 ) ) ;
#25627=CARTESIAN_POINT ( 'NONE',  ( 14.70517680308578790, -282.7847647462911596, -216.2876277470288926 ) ) ;
#25628=CARTESIAN_POINT ( 'NONE',  ( -29.84099491404666082, -274.3113054987382498, -193.7273171777334824 ) ) ;
#25629=CARTESIAN_POINT ( 'NONE',  ( -70.30294375176407584, -277.3078857283183538, -339.9640346678647234 ) ) ;
#25630=CARTESIAN_POINT ( 'NONE',  ( -41.08769931505037931, -297.0197877011902392, -344.7196237511550407 ) ) ;
#25633=CARTESIAN_POINT ( 'NONE',  ( -72.68301609920166584, -295.7292325444900030, -203.2860891920712163 ) ) ;
#25634=CARTESIAN_POINT ( 'NONE',  ( -32.42267340908522044, -276.4962532529142436, -343.3068851284983793 ) ) ;
#25635=CARTESIAN_POINT ( 'NONE',  ( -37.62039264774393388, -299.1284046588111210, -193.6707350009189668 ) ) ;
#25636=CARTESIAN_POINT ( 'NONE',  ( -19.59428103012816180, -288.0436757755916233, -198.5070775513977424 ) ) ;
#25638=CARTESIAN_POINT ( 'NONE',  ( -111.2918881712147368, -297.8340676649014540, -289.2307598041940082 ) ) ;
#25639=CARTESIAN_POINT ( 'NONE',  ( -30.61047808688418925, -296.1738977209472523, -346.6677321666859370 ) ) ;
#25640=CARTESIAN_POINT ( 'NONE',  ( -109.1618181126651592, -292.8241350131525564, -249.2941676546431040 ) ) ;
#25641=CARTESIAN_POINT ( 'NONE',  ( -4.737268542336128263, -278.4824537626984124, -203.0040138855710552 ) ) ;
#25642=CARTESIAN_POINT ( 'NONE',  ( -75.25995026235231933, -281.4631024603752962, -206.2431335187117440 ) ) ;
#25643=CARTESIAN_POINT ( 'NONE',  ( -111.9865001276048986, -270.5725786021788508, -270.3359667857977229 ) ) ;
#25644=CARTESIAN_POINT ( 'NONE',  ( -11.10714175854606189, -284.5743800810157609, -341.4946611779132013 ) ) ;
#25645=CARTESIAN_POINT ( 'NONE',  ( 20.59335882061688139, -285.8424798724951756, -225.4416899004503421 ) ) ;
#25646=CARTESIAN_POINT ( 'NONE',  ( -54.56600731238864910, -170.2994449650265096, -364.0860178467487458 ) ) ;
#25648=CARTESIAN_POINT ( 'NONE',  ( -30.52508452115705495, -285.8072984000240240, -197.6080265558017288 ) ) ;
#25650=CARTESIAN_POINT ( 'NONE',  ( -24.57146089363258312, -283.9726479932963343, -346.0352106241145407 ) ) ;
#25651=CARTESIAN_POINT ( 'NONE',  ( -34.48319489723353826, -298.5812350648678262, -197.2993321103043911 ) ) ;
#25652=CARTESIAN_POINT ( 'NONE',  ( -33.73061514378654380, -284.8915767187771735, -193.8433502127151087 ) ) ;
#25653=CARTESIAN_POINT ( 'NONE',  ( 34.10102936607029989, -282.1346251684736899, -242.1312818794532404 ) ) ;
#25655=CARTESIAN_POINT ( 'NONE',  ( -99.69372176527166118, -280.6595780536233065, -226.3732429364199277 ) ) ;
#25656=CARTESIAN_POINT ( 'NONE',  ( 21.04729040431934450, -281.2079403954513737, -220.1766455182886375 ) ) ;
#25658=CARTESIAN_POINT ( 'NONE',  ( -82.13390479932374433, -281.1952119285918457, -326.4764044574609443 ) ) ;
#25659=CARTESIAN_POINT ( 'NONE',  ( 202.9216279488346686, 293.3251575386738068, -83.23662280983118933 ) ) ;
#25661=CARTESIAN_POINT ( 'NONE',  ( 10.86399985531348733, -278.3837087097922449, -327.5995570998625226 ) ) ;
#25662=CARTESIAN_POINT ( 'NONE',  ( -90.69729355805023374, -230.0588105309422247, -347.5619421900863699 ) ) ;
#25664=CARTESIAN_POINT ( 'NONE',  ( 36.66691670201128517, -279.4418272682470956, -260.2510634191229997 ) ) ;
#25665=CARTESIAN_POINT ( 'NONE',  ( -16.92077093663188592, -294.0724854820045380, -197.1698639799152204 ) ) ;
#25666=CARTESIAN_POINT ( 'NONE',  ( -92.27274552457252810, -295.2131824268811897, -318.5946428386462230 ) ) ;
#25667=CARTESIAN_POINT ( 'NONE',  ( -34.95603508188709441, -291.5889850733971116, -193.4465122751517185 ) ) ;
#25670=CARTESIAN_POINT ( 'NONE',  ( -111.6967567103062322, -295.3487716004134427, -252.7562363852289309 ) ) ;
#25671=CARTESIAN_POINT ( 'NONE',  ( -3.012198179119665920, -286.9908707911066585, -335.7470691259181876 ) ) ;
#25672=CARTESIAN_POINT ( 'NONE',  ( 9.017714892348468680, -296.2690157128162127, -328.4071112095504645 ) ) ;
#25674=CARTESIAN_POINT ( 'NONE',  ( -109.4158608333471960, -286.0556496217638482, -255.9889630330912098 ) ) ;
#25676=CARTESIAN_POINT ( 'NONE',  ( 29.37612370723951472, -294.9891731240032300, -308.4363064969310244 ) ) ;
#25677=CARTESIAN_POINT ( 'NONE',  ( 29.37321052148537959, -282.4467158442050732, -300.2697392283906197 ) ) ;
#25678=CARTESIAN_POINT ( 'NONE',  ( -58.75511502022377641, -294.1179092739052408, -343.9655358312071485 ) ) ;
#25679=CARTESIAN_POINT ( 'NONE',  ( -111.3836305162620448, -291.0970844283563679, -290.9025727797135801 ) ) ;
#25680=CARTESIAN_POINT ( 'NONE',  ( -50.56194987510324523, -292.3799901568387440, -194.5669763903573255 ) ) ;
#25681=CARTESIAN_POINT ( 'NONE',  ( -88.65956010366774365, -289.9639465690058842, -322.2791038065706744 ) ) ;
#25683=CARTESIAN_POINT ( 'NONE',  ( -89.87931010611180227, -272.1253713169422781, -214.5409756786795299 ) ) ;
#25684=CARTESIAN_POINT ( 'NONE',  ( -27.51497411582626995, -279.2386571564418887, -197.7367365232332190 ) ) ;
#25685=EDGE_LOOP ( 'NONE', ( #23096, #77736 ) ) ;
#25686=CARTESIAN_POINT ( 'NONE',  ( -2.579733554756037606, -274.0070829431385846, -201.7087357506077581 ) ) ;
#25687=CARTESIAN_POINT ( 'NONE',  ( 18.37777377432308512, -278.1015011621257713, -319.4333934114329168 ) ) ;
#25688=CARTESIAN_POINT ( 'NONE',  ( -18.94295532091393497, -272.4309482982852728, -198.3887362015445603 ) ) ;
#25689=CARTESIAN_POINT ( 'NONE',  ( -105.1348051114124047, -298.1323903834429530, -242.2323885310863432 ) ) ;
#25690=CARTESIAN_POINT ( 'NONE',  ( -35.82125369465582310, -299.1512985992672498, -197.0517164500904812 ) ) ;
#25691=FACE_OUTER_BOUND ( 'NONE', #22296, .T. ) ;
#25692=CARTESIAN_POINT ( 'NONE',  ( -112.3552029044302998, -298.3215523385778170, -256.9665363251803569 ) ) ;
#25693=CARTESIAN_POINT ( 'NONE',  ( 73.04948978576122443, -297.4307250721599871, -195.2319741477500656 ) ) ;
#25694=CARTESIAN_POINT ( 'NONE',  ( 21.88242546706848657, -293.6046374159868151, -227.4866480982354915 ) ) ;
#25695=CARTESIAN_POINT ( 'NONE',  ( -12.04070959418731235, -290.9625677101679457, -201.2037262385670999 ) ) ;
#25697=CARTESIAN_POINT ( 'NONE',  ( -13.08783334611800164, -274.8513833894338632, -197.3455247901048324 ) ) ;
#25698=CARTESIAN_POINT ( 'NONE',  ( -109.5830769536326414, -272.8618616679830780, -259.5187654142159204 ) ) ;
#25699=CARTESIAN_POINT ( 'NONE',  ( -8.641469825694837681, -284.6584747970617286, -340.0921619764920933 ) ) ;
#25700=CARTESIAN_POINT ( 'NONE',  ( -27.45254589757167807, -281.6139772762828102, -346.2791674358736032 ) ) ;
#25701=CARTESIAN_POINT ( 'NONE',  ( -97.85383888099049443, -277.2655848536886083, -317.8120805722413706 ) ) ;
#25703=CARTESIAN_POINT ( 'NONE',  ( -93.55268387274327324, -283.0863259365150384, -317.1898168104737010 ) ) ;
#25704=CARTESIAN_POINT ( 'NONE',  ( 37.45113411599673015, -279.6543336534976447, -278.3496193524680962 ) ) ;
#25705=CARTESIAN_POINT ( 'NONE',  ( 1.164400433653314249, -275.1022051699037547, -333.1318705715253259 ) ) ;
#25706=CARTESIAN_POINT ( 'NONE',  ( -95.65078582317094913, -279.9027245443101037, -317.5515851221219350 ) ) ;
#25709=CARTESIAN_POINT ( 'NONE',  ( -9.549216625494851840, -296.6354199188683083, -194.3826371356322795 ) ) ;
#25710=CARTESIAN_POINT ( 'NONE',  ( -109.9664595759330155, -280.8014833033493005, -250.9290821974932157 ) ) ;
#25712=CARTESIAN_POINT ( 'NONE',  ( -67.28773519107451762, -285.3619353537811776, -339.7336571039463706 ) ) ;
#25714=CARTESIAN_POINT ( 'NONE',  ( 14.60772790238195107, -286.3212544238138548, -324.5266233820272532 ) ) ;
#25716=CARTESIAN_POINT ( 'NONE',  ( -71.12716255693898404, -294.3033585865081250, -335.5340088935061544 ) ) ;
#25717=CARTESIAN_POINT ( 'NONE',  ( -37.29055519897222837, -287.1910898083224879, -344.5963041702376017 ) ) ;
#25718=CARTESIAN_POINT ( 'NONE',  ( -49.37856652629597676, -155.6656457446864010, -366.7448178265262868 ) ) ;
#25719=CARTESIAN_POINT ( 'NONE',  ( -94.62602932240814368, -293.8822009894938105, -318.7907966750074706 ) ) ;
#25720=CARTESIAN_POINT ( 'NONE',  ( -78.13531591035727786, -283.9940897731921154, -205.8739978481109176 ) ) ;
#25721=CARTESIAN_POINT ( 'NONE',  ( 34.10306240125144939, -283.3943974560218635, -288.9070856567997794 ) ) ;
#25722=CARTESIAN_POINT ( 'NONE',  ( -44.34840006887846187, -281.3793482781901503, -346.0767118028122127 ) ) ;
#25723=CARTESIAN_POINT ( 'NONE',  ( -102.8454316650584275, -290.1155329157977576, -302.5831780459953961 ) ) ;
#25724=CARTESIAN_POINT ( 'NONE',  ( -34.30705430493454600, -281.5162894098867810, -196.8218395327261590 ) ) ;
#25725=CARTESIAN_POINT ( 'NONE',  ( -7.943923662102324812, -281.2502555535783699, -203.3520995798398587 ) ) ;
#25726=CARTESIAN_POINT ( 'NONE',  ( 21.14485214991424655, -290.1835821195315361, -317.8970111168432595 ) ) ;
#25729=CARTESIAN_POINT ( 'NONE',  ( -58.12161569055139410, -273.7909900291650729, -196.1626211770820305 ) ) ;
#25731=CARTESIAN_POINT ( 'NONE',  ( -111.0390911448227200, -292.3780697433153364, -282.2963611797865724 ) ) ;
#25733=CARTESIAN_POINT ( 'NONE',  ( -88.52914483777347243, -293.9090924074131408, -206.2264541496106460 ) ) ;
#25735=CARTESIAN_POINT ( 'NONE',  ( -17.85824711556551492, -274.8013122890735076, -342.9588003310910835 ) ) ;
#25737=CARTESIAN_POINT ( 'NONE',  ( -30.68138555019360680, -293.3691461168232308, -346.2694879088334119 ) ) ;
#25738=CARTESIAN_POINT ( 'NONE',  ( -63.33522389967379240, -273.0529365769760943, -202.0231641902481385 ) ) ;
#25739=CARTESIAN_POINT ( 'NONE',  ( -76.21822789854435598, -291.1022548893236603, -332.9656173455052794 ) ) ;
#25740=CARTESIAN_POINT ( 'NONE',  ( 30.24888643064024052, -283.7143058662104522, -300.6447381919217605 ) ) ;
#25742=CARTESIAN_POINT ( 'NONE',  ( -106.7330034028650800, -292.3912392892430603, -238.2435322501283110 ) ) ;
#25743=CARTESIAN_POINT ( 'NONE',  ( -110.7636443102908714, -292.1388055199153087, -248.8549238591254777 ) ) ;
#25744=CARTESIAN_POINT ( 'NONE',  ( -57.65290562738642421, -291.6159439643503219, -200.1908048483340679 ) ) ;
#25745=CARTESIAN_POINT ( 'NONE',  ( -105.3084130313718987, -286.9705025652195900, -238.5278767630905463 ) ) ;
#25746=CARTESIAN_POINT ( 'NONE',  ( -53.76254813612103334, -280.0138378833462411, -195.0778590257286282 ) ) ;
#25747=CARTESIAN_POINT ( 'NONE',  ( -105.2090043722127461, -295.0666929450824227, -237.1445075327571033 ) ) ;
#25748=CARTESIAN_POINT ( 'NONE',  ( 6.923273902218037179, -282.3015927835048728, -333.4311748372482498 ) ) ;
#25749=CARTESIAN_POINT ( 'NONE',  ( 36.60642713423293770, -277.3207133737288927, -263.2797449635788212 ) ) ;
#25750=CARTESIAN_POINT ( 'NONE',  ( -37.37352853689063181, -282.5519495502701375, -200.3611179825600459 ) ) ;
#25751=CARTESIAN_POINT ( 'NONE',  ( -72.29229894553861868, -275.6490838595548212, -337.5973187841282765 ) ) ;
#25753=CARTESIAN_POINT ( 'NONE',  ( -95.16898982769096449, -283.4314139382817075, -315.0356911304073151 ) ) ;
#25754=CARTESIAN_POINT ( 'NONE',  ( -110.1769558053102003, -280.0591821721940278, -246.4643133719727643 ) ) ;
#25755=CARTESIAN_POINT ( 'NONE',  ( 32.50294254440365194, -286.2010408273715711, -238.3811718237456034 ) ) ;
#25756=CARTESIAN_POINT ( 'NONE',  ( 13.58438430990091561, -294.5375101294663409, -216.6535027333626999 ) ) ;
#25757=CARTESIAN_POINT ( 'NONE',  ( 29.23851005349852983, -276.6655694952522140, -233.1916905835554132 ) ) ;
#25758=CARTESIAN_POINT ( 'NONE',  ( 37.45967281773607738, -276.6643435583600308, -254.2352225771534222 ) ) ;
#25759=CARTESIAN_POINT ( 'NONE',  ( -109.1317158414841799, -278.5600772795537523, -257.1250442297024961 ) ) ;
#25760=CARTESIAN_POINT ( 'NONE',  ( -111.5577648836208766, -298.6807984470532915, -260.3767669189888920 ) ) ;
#25762=CARTESIAN_POINT ( 'NONE',  ( -96.38832024477478910, -283.1841407755607065, -224.3672283150072246 ) ) ;
#25763=CARTESIAN_POINT ( 'NONE',  ( -8.515197623694632512, -292.0860370985155328, -198.9834110643347174 ) ) ;
#25764=CARTESIAN_POINT ( 'NONE',  ( 35.19255307683887679, -289.4489897864291947, -293.7111185641127236 ) ) ;
#25765=CARTESIAN_POINT ( 'NONE',  ( -2.279549647253553690, -291.4480219074775391, -205.9661836086507094 ) ) ;
#25767=CARTESIAN_POINT ( 'NONE',  ( -83.89289766830796680, -290.0019943030525269, -209.7007780552170857 ) ) ;
#25768=CARTESIAN_POINT ( 'NONE',  ( -37.54574934532697483, -291.7162823329366574, -197.3278115807005122 ) ) ;
#25769=VERTEX_POINT ( 'NONE', #12945 ) ;
#25770=CARTESIAN_POINT ( 'NONE',  ( -102.0330907817240131, -291.0886148197743637, -311.6476078826511298 ) ) ;
#25771=CARTESIAN_POINT ( 'NONE',  ( -91.31530743669969752, -279.5904776051542058, -221.1784258958365683 ) ) ;
#25772=CARTESIAN_POINT ( 'NONE',  ( -110.0570086449736067, -295.1643557943131100, -294.7327493761372921 ) ) ;
#25773=CARTESIAN_POINT ( 'NONE',  ( -89.82274634191698226, -285.9862872428379319, -214.0832377296034679 ) ) ;
#25774=CARTESIAN_POINT ( 'NONE',  ( -15.42354209600849480, -286.6614657292587367, -196.5132041097130013 ) ) ;
#25775=CARTESIAN_POINT ( 'NONE',  ( -105.2320262026618423, -284.5242119666446570, -297.3872320343882620 ) ) ;
#25776=CARTESIAN_POINT ( 'NONE',  ( 203.3289701366145152, 295.9433977242509286, -68.67267355934257012 ) ) ;
#25778=CARTESIAN_POINT ( 'NONE',  ( 120.1291425852486583, 149.7169047988457748, -262.4347193084595347 ) ) ;
#25779=CARTESIAN_POINT ( 'NONE',  ( 24.90698337435117793, -23.76329158025230015, -341.4199860761482341 ) ) ;
#25780=CARTESIAN_POINT ( 'NONE',  ( -4.022037595628576767, -273.7004142286585306, -205.2133306798716035 ) ) ;
#25781=CARTESIAN_POINT ( 'NONE',  ( -18.95262775744699013, -275.7301201017140215, -341.3263777229997231 ) ) ;
#25782=CARTESIAN_POINT ( 'NONE',  ( -48.95450548983835404, -297.4157943772210047, -194.2504790863257256 ) ) ;
#25783=CARTESIAN_POINT ( 'NONE',  ( 174.6243218329550757, 240.3365076134214178, -177.4484248103281061 ) ) ;
#25785=CARTESIAN_POINT ( 'NONE',  ( 30.81858792213831677, -273.7865838961465101, -235.6123999579116344 ) ) ;
#25786=CARTESIAN_POINT ( 'NONE',  ( -35.38570508461067732, -275.8371450463314432, -196.3609527273910373 ) ) ;
#25787=CARTESIAN_POINT ( 'NONE',  ( -113.5570086104289658, -273.7388997161712609, -261.8335589948311508 ) ) ;
#25788=CARTESIAN_POINT ( 'NONE',  ( -74.74202174047974268, -290.0568641876849938, -333.1388978529938640 ) ) ;
#25789=CARTESIAN_POINT ( 'NONE',  ( -79.38005676511495778, -296.4071618938556298, -334.6801306571198893 ) ) ;
#25790=CARTESIAN_POINT ( 'NONE',  ( -113.5907721819394141, -296.9109925778882371, -281.0275484406095643 ) ) ;
#25791=CARTESIAN_POINT ( 'NONE',  ( -50.46912369117863051, -295.3911572754605004, -342.1710807668425787 ) ) ;
#25793=CARTESIAN_POINT ( 'NONE',  ( -37.10642829824096367, -278.9693415054871934, -345.9335705797932974 ) ) ;
#25796=CARTESIAN_POINT ( 'NONE',  ( -42.41972680664798645, -279.4973746876558494, -193.5904168764288613 ) ) ;
#25797=CARTESIAN_POINT ( 'NONE',  ( 16.71289508835151238, -277.2000932482852136, -319.7914558029112868 ) ) ;
#25798=CARTESIAN_POINT ( 'NONE',  ( 25.24516168202696065, -277.8897785374628597, -313.5435093532957467 ) ) ;
#25800=CARTESIAN_POINT ( 'NONE',  ( -109.1081219787577368, -276.2751154481544518, -293.5072813455016103 ) ) ;
#25801=CARTESIAN_POINT ( 'NONE',  ( -32.69337472332519212, -274.6046302645801234, -197.4350603189898266 ) ) ;
#25802=CARTESIAN_POINT ( 'NONE',  ( -92.27273266985599776, -295.8215530872476506, -221.3921831174093029 ) ) ;
#25804=CARTESIAN_POINT ( 'NONE',  ( -93.94187354024062131, -279.3714059192312789, -224.2588363226474257 ) ) ;
#25805=CARTESIAN_POINT ( 'NONE',  ( -37.51737777987461442, -287.7391046918958750, -346.8807552776460170 ) ) ;
#25806=CARTESIAN_POINT ( 'NONE',  ( -60.28419677691929479, -275.7550055324873028, -198.9021465559121680 ) ) ;
#25808=CARTESIAN_POINT ( 'NONE',  ( -109.9510235274600376, -289.6312277285310870, -279.3326218908130159 ) ) ;
#25809=CARTESIAN_POINT ( 'NONE',  ( -110.1308739028959138, -283.5878546670392097, -295.1612987813265363 ) ) ;
#25810=CARTESIAN_POINT ( 'NONE',  ( 34.09748294977161009, -279.5393322973619661, -250.9627124732487005 ) ) ;
#25811=CARTESIAN_POINT ( 'NONE',  ( 33.30530965296356527, -279.8565443958207766, -249.7607556845141801 ) ) ;
#25812=CARTESIAN_POINT ( 'NONE',  ( -75.43643540319085616, -283.6196787863938198, -206.4071865780526878 ) ) ;
#25813=CARTESIAN_POINT ( 'NONE',  ( 24.80478984558882871, -288.9832002199053704, -228.2840840740589101 ) ) ;
#25814=CARTESIAN_POINT ( 'NONE',  ( -94.25811432216426056, -280.4096335186494571, -224.0183483046573940 ) ) ;
#25816=CARTESIAN_POINT ( 'NONE',  ( -4.227951794944921460, -294.4888015480337344, -203.0529764801314911 ) ) ;
#25817=CARTESIAN_POINT ( 'NONE',  ( -45.14669500603307739, -278.1945928290650727, -194.7240645622421198 ) ) ;
#25818=CARTESIAN_POINT ( 'NONE',  ( 20.92318118658734605, -276.8231024925980250, -314.5096884450998687 ) ) ;
#25819=CARTESIAN_POINT ( 'NONE',  ( -63.25549200618215195, -285.3891191476989775, -340.9196314062497777 ) ) ;
#25821=CARTESIAN_POINT ( 'NONE',  ( -110.8558847328221191, -292.2490257316667908, -287.8800493199952371 ) ) ;
#25822=CARTESIAN_POINT ( 'NONE',  ( -73.90191560405894222, -293.5375007154946161, -335.8610894536354294 ) ) ;
#25823=CARTESIAN_POINT ( 'NONE',  ( 29.99499273372738628, -286.2677321309743661, -233.2381440699909945 ) ) ;
#25824=CARTESIAN_POINT ( 'NONE',  ( -92.25494350317529779, -289.6502297942929545, -221.0372926380688909 ) ) ;
#25826=CARTESIAN_POINT ( 'NONE',  ( 32.98344197680759038, -274.5182354711825496, -291.7499168344537566 ) ) ;
#25827=CARTESIAN_POINT ( 'NONE',  ( -17.91977323886857931, -292.9386378800824673, -342.0106415929492414 ) ) ;
#25830=CARTESIAN_POINT ( 'NONE',  ( -50.42824481119912150, -290.3678449910482300, -195.1849907922274667 ) ) ;
#25831=CARTESIAN_POINT ( 'NONE',  ( -46.84789082344370570, -287.5297181109634721, -197.1245903374295381 ) ) ;
#25832=CARTESIAN_POINT ( 'NONE',  ( 23.31954395817320957, -286.4095506278797529, -316.1234112176571216 ) ) ;
#25833=CARTESIAN_POINT ( 'NONE',  ( -110.9070211703337208, -285.9339657820697767, -273.6826870961493228 ) ) ;
#25835=CARTESIAN_POINT ( 'NONE',  ( -87.81327407348437930, -286.1273977716414834, -217.3967719548230662 ) ) ;
#25836=CARTESIAN_POINT ( 'NONE',  ( 5.539117145922015872, -294.6096153730299534, -208.3962706065396731 ) ) ;
#25837=CARTESIAN_POINT ( 'NONE',  ( -110.7815009478636057, -276.4047906252646385, -288.1892350526958353 ) ) ;
#25838=CARTESIAN_POINT ( 'NONE',  ( 37.57227483734749285, -276.1076319789668787, -288.1278113834255805 ) ) ;
#25839=CARTESIAN_POINT ( 'NONE',  ( 8.006600369479306423, -290.7459360878327743, -209.8570237530543920 ) ) ;
#25840=CARTESIAN_POINT ( 'NONE',  ( -114.3849019319820002, -278.5365532289854400, -271.6083964946004130 ) ) ;
#25841=CARTESIAN_POINT ( 'NONE',  ( -111.4339917909207429, -298.4097718335198124, -279.8391550080929733 ) ) ;
#25844=CARTESIAN_POINT ( 'NONE',  ( -89.97807872487524605, -275.9444495014743666, -322.7817942617505196 ) ) ;
#25845=CARTESIAN_POINT ( 'NONE',  ( 27.56872345658622336, -279.0503911176733709, -232.7893525645756938 ) ) ;
#25847=CARTESIAN_POINT ( 'NONE',  ( 36.61804261008658301, -273.7949141879465742, -251.5817620615348744 ) ) ;
#25848=CARTESIAN_POINT ( 'NONE',  ( -35.61514498691887098, -296.5502584981659879, -344.0468399903400609 ) ) ;
#25849=CARTESIAN_POINT ( 'NONE',  ( 25.66848100500453356, -281.0526126696997835, -314.1015914732294618 ) ) ;
#25850=CARTESIAN_POINT ( 'NONE',  ( -71.02839428366141306, -296.4493392220763894, -335.4029488731391666 ) ) ;
#25851=CARTESIAN_POINT ( 'NONE',  ( -113.4509216657957182, -297.7692705867122527, -278.1511544995717031 ) ) ;
#25852=CARTESIAN_POINT ( 'NONE',  ( -93.79202054805612931, -272.8750204820507861, -224.0225782304559345 ) ) ;
#25853=CARTESIAN_POINT ( 'NONE',  ( -64.82765207447191358, -293.6933763777807940, -200.5652437169594293 ) ) ;
#25854=CARTESIAN_POINT ( 'NONE',  ( 25.54387905179369156, -287.1305618508691850, -225.9041207761447652 ) ) ;
#25855=CARTESIAN_POINT ( 'NONE',  ( 36.69353084813054267, -273.8970994999799586, -286.5179221841542017 ) ) ;
#25856=CARTESIAN_POINT ( 'NONE',  ( -1.802610534173727741, -288.4277567463471428, -338.6690466245649986 ) ) ;
#25857=CARTESIAN_POINT ( 'NONE',  ( 28.43384978605038071, -287.0457024460403659, -302.5633769229399945 ) ) ;
#25858=CARTESIAN_POINT ( 'NONE',  ( -111.3896078978784061, -288.3990361931747657, -282.2736326078452862 ) ) ;
#25860=CARTESIAN_POINT ( 'NONE',  ( 202.9738562182569694, 296.4636489450776367, -53.99999999999997868 ) ) ;
#25861=CARTESIAN_POINT ( 'NONE',  ( 8.013246788581509961, -287.9202810026690145, -327.6404094554928861 ) ) ;
#25864=CARTESIAN_POINT ( 'NONE',  ( -69.07820186173226773, -284.4006734740404454, -340.2726589327171496 ) ) ;
#25865=CARTESIAN_POINT ( 'NONE',  ( 38.62085226948885008, -292.4675736104839530, -258.9356181331404514 ) ) ;
#25866=CARTESIAN_POINT ( 'NONE',  ( -33.97126039139428144, -281.6940120787344881, -194.2356915295061697 ) ) ;
#25867=CARTESIAN_POINT ( 'NONE',  ( -53.67165624039790828, -281.1621470493041102, -195.5631285387612195 ) ) ;
#25868=CARTESIAN_POINT ( 'NONE',  ( -8.496194895253452728, -282.4970530477719990, -337.4203219174742117 ) ) ;
#25869=CARTESIAN_POINT ( 'NONE',  ( -57.10327281808218203, -279.3071096973661156, -342.7647609468566543 ) ) ;
#25870=CARTESIAN_POINT ( 'NONE',  ( -112.3058002325742706, -296.3314603799390738, -288.0074543607191799 ) ) ;
#25871=CARTESIAN_POINT ( 'NONE',  ( -98.71533538762201943, -287.9931263058210220, -312.8703315742963014 ) ) ;
#25872=CARTESIAN_POINT ( 'NONE',  ( -63.17557711464727532, -296.6280401393570969, -201.7010257756815008 ) ) ;
#25874=ORIENTED_EDGE ( 'NONE', *, *, #58963, .F. ) ;
#25876=CARTESIAN_POINT ( 'NONE',  ( -110.9179070595490089, -286.3217628247462585, -281.9984686515474550 ) ) ;
#25877=CARTESIAN_POINT ( 'NONE',  ( -71.92229973248871033, -296.5782507635937009, -338.8131058422523552 ) ) ;
#25878=CARTESIAN_POINT ( 'NONE',  ( -109.9730360505223246, -285.0887293693722881, -279.0787349729150719 ) ) ;
#25880=CARTESIAN_POINT ( 'NONE',  ( -41.38407786455062620, -276.1606034625448274, -347.0324849042550568 ) ) ;
#25881=CARTESIAN_POINT ( 'NONE',  ( -113.9061788668451953, -291.3000616905659967, -262.6554331680857217 ) ) ;
#25882=CARTESIAN_POINT ( 'NONE',  ( -40.73701479434670603, -284.1495964752608074, -194.6210743333838877 ) ) ;
#25883=CARTESIAN_POINT ( 'NONE',  ( -74.67236002090217539, -291.9025490433749610, -203.0397534426279833 ) ) ;
#25884=CARTESIAN_POINT ( 'NONE',  ( -69.97808810469915386, -289.8275995896190125, -335.6969039014205123 ) ) ;
#25887=CARTESIAN_POINT ( 'NONE',  ( -12.12095700411519239, -92.64272014086816398, -356.3117460650181556 ) ) ;
#25888=CARTESIAN_POINT ( 'NONE',  ( -87.84800523043182352, -285.2628329593632657, -327.6314872641165721 ) ) ;
#25889=CARTESIAN_POINT ( 'NONE',  ( 31.95455697924147032, -291.4809262143061233, -303.7686719486574702 ) ) ;
#25891=CARTESIAN_POINT ( 'NONE',  ( 17.82845731876507855, -281.1583948601936527, -318.6361612399400087 ) ) ;
#25892=CARTESIAN_POINT ( 'NONE',  ( -31.45611935868447517, -276.6466098803346085, -347.1672559327260501 ) ) ;
#25893=CARTESIAN_POINT ( 'NONE',  ( -110.6891459279048036, -280.7440893819315306, -255.4581790320177390 ) ) ;
#25894=CARTESIAN_POINT ( 'NONE',  ( 47.06908910409267577, 10.77964184115877444, -330.2742531180653600 ) ) ;
#25895=CARTESIAN_POINT ( 'NONE',  ( 35.61852786047657560, -279.8394870554832892, -247.6584435863159683 ) ) ;
#25896=CARTESIAN_POINT ( 'NONE',  ( -69.46032988677893627, -283.6474778697021293, -202.9657143351045931 ) ) ;
#25897=CARTESIAN_POINT ( 'NONE',  ( -94.17585406997072539, -275.1019723504455214, -220.2593772175699200 ) ) ;
#25898=CARTESIAN_POINT ( 'NONE',  ( -98.78165813105036364, -296.4966903541272245, -309.9900991268975190 ) ) ;
#25900=CARTESIAN_POINT ( 'NONE',  ( -0.9983329195906816000, -291.2301665409301563, -206.4685099808981761 ) ) ;
#25901=CARTESIAN_POINT ( 'NONE',  ( 21.65776030399775820, -276.8681311117747441, -319.6802466823783675 ) ) ;
#25902=CARTESIAN_POINT ( 'NONE',  ( 5.176745952576675691, -274.6449562451687711, -210.9590948345535537 ) ) ;
#25903=CARTESIAN_POINT ( 'NONE',  ( 4.705225719283427033, -273.5255036196151650, -206.1611522513642001 ) ) ;
#25905=CARTESIAN_POINT ( 'NONE',  ( -73.39312330142507790, -271.5741868509902588, -204.5368220061378679 ) ) ;
#25909=CARTESIAN_POINT ( 'NONE',  ( -34.82220260114848998, -284.0994702711495279, -343.6394122138794955 ) ) ;
#25910=CARTESIAN_POINT ( 'NONE',  ( 13.02609450617649856, -284.1204937703224687, -327.3263356395374331 ) ) ;
#25911=CARTESIAN_POINT ( 'NONE',  ( -108.7627168652007015, -284.1068285045616904, -254.7164616514315867 ) ) ;
#25912=CARTESIAN_POINT ( 'NONE',  ( -5.954693553600145073, -275.0324268516998245, -337.1679706702036583 ) ) ;
#25913=CARTESIAN_POINT ( 'NONE',  ( 33.41576028726181136, -283.7072990443342633, -292.9841591951132500 ) ) ;
#25914=CARTESIAN_POINT ( 'NONE',  ( -91.49033523150968961, -276.3202306914116662, -320.4216960292102954 ) ) ;
#25915=CARTESIAN_POINT ( 'NONE',  ( 82.64890176555634582, -299.5541904835127980, -195.3611179825600175 ) ) ;
#25916=CARTESIAN_POINT ( 'NONE',  ( 24.04485864437597442, -276.0788496436803712, -230.2872302795820190 ) ) ;
#25918=CARTESIAN_POINT ( 'NONE',  ( -90.95284487861292178, -280.1175249442051722, -215.2414600216427800 ) ) ;
#25923=CARTESIAN_POINT ( 'NONE',  ( -98.36372191485419592, -287.0198539397164268, -225.3679876411632392 ) ) ;
#25924=CARTESIAN_POINT ( 'NONE',  ( -80.25774089342543505, -294.8475509580432572, -329.6132501932872287 ) ) ;
#25925=CARTESIAN_POINT ( 'NONE',  ( -78.08943754177407470, -288.9328766953452146, -335.6377647308412975 ) ) ;
#25926=CARTESIAN_POINT ( 'NONE',  ( 36.46049290610081783, -285.8730302373453469, -276.5886039220040402 ) ) ;
#25927=CARTESIAN_POINT ( 'NONE',  ( 24.03546739342869643, -285.5670452915640567, -229.6705733914454299 ) ) ;
#25928=CARTESIAN_POINT ( 'NONE',  ( -90.52915840012502713, -289.5256324248924784, -218.8920175849421526 ) ) ;
#25929=CARTESIAN_POINT ( 'NONE',  ( -91.02145377976198404, -285.0412516402019492, -320.4172320241023044 ) ) ;
#25930=CARTESIAN_POINT ( 'NONE',  ( 35.99526119829556592, -273.3495455935378118, -254.5939179653592817 ) ) ;
#25931=CARTESIAN_POINT ( 'NONE',  ( -32.33838369109098920, -284.5140983906240422, -194.3125229451406710 ) ) ;
#25932=CARTESIAN_POINT ( 'NONE',  ( -33.48931516368976702, -300.1005329123065053, -195.3597958697542651 ) ) ;
#25933=CARTESIAN_POINT ( 'NONE',  ( 32.33313569441546065, -285.9204056174309585, -298.7032872206346497 ) ) ;
#25934=AXIS2_PLACEMENT_3D ( 'NONE', #18318, #11215, #32992 ) ;
#25935=CARTESIAN_POINT ( 'NONE',  ( -27.53870865084137520, -281.1208579356245423, -197.7335285178276933 ) ) ;
#25936=CARTESIAN_POINT ( 'NONE',  ( -23.62097655468325286, -290.8774919726514554, -344.3177367053257854 ) ) ;
#25939=CARTESIAN_POINT ( 'NONE',  ( -109.4186868777834576, -298.1814181051570927, -293.0808471850168644 ) ) ;
#25941=CARTESIAN_POINT ( 'NONE',  ( -24.50983114626673753, -278.2157762165726353, -196.4669789422241024 ) ) ;
#25942=CARTESIAN_POINT ( 'NONE',  ( 30.76055634303483188, -292.2879753756741366, -234.6622587821045443 ) ) ;
#25943=CARTESIAN_POINT ( 'NONE',  ( -97.06771932712487683, -294.3516957407734935, -313.7329324393978141 ) ) ;
#25944=CARTESIAN_POINT ( 'NONE',  ( 34.82164466854323592, -280.0537429082800713, -256.3773019793481467 ) ) ;
#25945=CARTESIAN_POINT ( 'NONE',  ( -16.20889725241792334, -272.4071833189682366, -198.9300645962699718 ) ) ;
#25946=CARTESIAN_POINT ( 'NONE',  ( 30.30313881440716273, -294.4826289100929557, -241.5008806847925769 ) ) ;
#25947=CARTESIAN_POINT ( 'NONE',  ( 10.59707575819634329, -295.1948066931273615, -210.1954327657594490 ) ) ;
#25948=CARTESIAN_POINT ( 'NONE',  ( -93.14239701790498316, -295.7487493848604458, -218.2361083365121885 ) ) ;
#25949=CARTESIAN_POINT ( 'NONE',  ( -25.09353482912474931, -293.1380283764050318, -345.4075125059563902 ) ) ;
#25950=CARTESIAN_POINT ( 'NONE',  ( -110.2038140223481264, -291.8412104281912889, -280.7706324348624207 ) ) ;
#25952=CARTESIAN_POINT ( 'NONE',  ( -34.86202760497246800, -292.8869309653617279, -197.2416749352204590 ) ) ;
#25954=CARTESIAN_POINT ( 'NONE',  ( -73.50919728821972399, -281.5492770470243613, -336.5277356159203919 ) ) ;
#25955=CARTESIAN_POINT ( 'NONE',  ( 34.21648972488689822, -293.3617048441598740, -255.9241700721964321 ) ) ;
#25956=CARTESIAN_POINT ( 'NONE',  ( -25.39559152602119596, -280.2004035161702404, -194.2934475221877619 ) ) ;
#25957=CARTESIAN_POINT ( 'NONE',  ( -92.42157317789884985, -283.4809958903768461, -324.1379891848655461 ) ) ;
#25958=CARTESIAN_POINT ( 'NONE',  ( -79.22099099712900738, -287.6181027501376093, -332.4408779614646505 ) ) ;
#25960=CARTESIAN_POINT ( 'NONE',  ( 33.93293379882927496, -280.3801847030492809, -297.6124355655138061 ) ) ;
#25961=CARTESIAN_POINT ( 'NONE',  ( 39.33131161188143210, -286.4516904057510942, -268.7052859836560401 ) ) ;
#25963=CARTESIAN_POINT ( 'NONE',  ( 29.12381975778757592, -295.5830270378971818, -302.5535620473963832 ) ) ;
#25964=CARTESIAN_POINT ( 'NONE',  ( 34.65196760190284664, -277.3048094974898845, -296.1202706597088650 ) ) ;
#25965=CARTESIAN_POINT ( 'NONE',  ( -76.82972323775312873, -279.1744091201867946, -208.8778553392625952 ) ) ;
#25966=CARTESIAN_POINT ( 'NONE',  ( 38.81685847085416441, -293.8608073330497064, -281.7133845686021232 ) ) ;
#25967=CARTESIAN_POINT ( 'NONE',  ( -93.34854435141173212, -281.9297358671645384, -321.1006031169986841 ) ) ;
#25968=CARTESIAN_POINT ( 'NONE',  ( 22.78795225624744702, -292.0298258460766760, -228.5319202577205999 ) ) ;
#25969=CARTESIAN_POINT ( 'NONE',  ( -86.14111594483458134, -295.3757364897904267, -213.3399077614377859 ) ) ;
#25972=CARTESIAN_POINT ( 'NONE',  ( 30.64052013739363645, -293.4190888271538142, -297.2652736617739606 ) ) ;
#25974=CARTESIAN_POINT ( 'NONE',  ( -37.30987171927208834, -289.5523547857346784, -200.3611179825600459 ) ) ;
#25975=CARTESIAN_POINT ( 'NONE',  ( -46.09112082227374430, -297.0024990591858227, -194.0966580412323879 ) ) ;
#25976=CARTESIAN_POINT ( 'NONE',  ( 37.20589397083265482, -279.8645778220592888, -283.9593905875534006 ) ) ;
#25977=CARTESIAN_POINT ( 'NONE',  ( -7.550713321903794295, -287.7496544439184163, -199.8364319631869819 ) ) ;
#25978=CARTESIAN_POINT ( 'NONE',  ( -13.28987695017997339, -288.5641777071908223, -339.2850601675242501 ) ) ;
#25980=CARTESIAN_POINT ( 'NONE',  ( -41.88012481404229703, -278.6304674994204333, -343.9272871104193996 ) ) ;
#25981=CARTESIAN_POINT ( 'NONE',  ( -110.6565072384489667, -294.7541120833667492, -256.2651225882140693 ) ) ;
#25982=CARTESIAN_POINT ( 'NONE',  ( -78.08829503046197829, -299.2566856577523708, -208.5120695833952595 ) ) ;
#25983=CARTESIAN_POINT ( 'NONE',  ( -106.8156270863670159, -277.6618542183446721, -246.5301755951784628 ) ) ;
#25985=CARTESIAN_POINT ( 'NONE',  ( -34.75605588228874154, -297.7504167085210725, -193.3824032948462843 ) ) ;
#25986=CARTESIAN_POINT ( 'NONE',  ( -64.32041632493388761, -291.3269781072776823, -339.7954894076447090 ) ) ;
#25987=CARTESIAN_POINT ( 'NONE',  ( 14.87497259471225597, -294.3732118444519301, -214.7922058508447094 ) ) ;
#25989=CARTESIAN_POINT ( 'NONE',  ( -109.2777500221154980, -291.0322660237165451, -283.3648633678579358 ) ) ;
#25991=EDGE_CURVE ( 'NONE', #39736, #8402, #70013, .T. ) ;
#25992=CARTESIAN_POINT ( 'NONE',  ( -114.2082137319480495, -297.2488066404342248, -266.7483527591360826 ) ) ;
#25993=CARTESIAN_POINT ( 'NONE',  ( -98.88106252421087561, -288.0961862353857441, -314.5785168999652228 ) ) ;
#25994=CARTESIAN_POINT ( 'NONE',  ( -35.83292491741726593, -298.4038377470325827, -193.3821790908798448 ) ) ;
#25998=CARTESIAN_POINT ( 'NONE',  ( -26.22625983952692152, -290.4332267996190353, -345.8538642469735009 ) ) ;
#25999=CARTESIAN_POINT ( 'NONE',  ( -55.56934967048406548, -297.7662352645559167, -350.3683826091709648 ) ) ;
#26000=CARTESIAN_POINT ( 'NONE',  ( -109.8102806463183470, -286.7926487064293042, -251.6974295125035042 ) ) ;
#26001=CARTESIAN_POINT ( 'NONE',  ( 19.17609989929905367, -286.8313636216280429, -321.8037927117418917 ) ) ;
#26002=CARTESIAN_POINT ( 'NONE',  ( -60.00726863166994463, -271.7577189236351387, -198.9885707427638124 ) ) ;
#26003=CARTESIAN_POINT ( 'NONE',  ( -104.5148179467219904, -274.8977431781710266, -238.2817408471631211 ) ) ;
#26005=CARTESIAN_POINT ( 'NONE',  ( -111.8076809284111874, -288.6573627805786373, -268.3998938313917506 ) ) ;
#26006=CARTESIAN_POINT ( 'NONE',  ( -102.5307339521301344, -279.9001831262722817, -309.0734714049813192 ) ) ;
#26008=CARTESIAN_POINT ( 'NONE',  ( -64.81611647204123017, -279.6830500953275873, -202.7286077041536601 ) ) ;
#26009=CARTESIAN_POINT ( 'NONE',  ( 9.348007857893522399, -280.0619235614337867, -214.0460021404753945 ) ) ;
#26010=CARTESIAN_POINT ( 'NONE',  ( -5.400930296626684779, -277.7213310088902745, -340.0839961038166166 ) ) ;
#26011=CARTESIAN_POINT ( 'NONE',  ( 5.972438054300714505, -279.4204340743924604, -207.1796796385847870 ) ) ;
#26012=CARTESIAN_POINT ( 'NONE',  ( 191.7941899171395050, 277.5480571852982621, -124.4921890884961044 ) ) ;
#26013=CARTESIAN_POINT ( 'NONE',  ( 30.34128672008207417, -276.9642122907782777, -306.6926298764308285 ) ) ;
#26017=CARTESIAN_POINT ( 'NONE',  ( 17.57702608577497827, -276.3395470037212931, -217.3075452942337620 ) ) ;
#26018=CARTESIAN_POINT ( 'NONE',  ( 31.95455697924148097, -295.6233781216988632, -236.9535640164627637 ) ) ;
#26021=CARTESIAN_POINT ( 'NONE',  ( 32.56422592585744979, -288.3399062829817012, -248.2422612819088386 ) ) ;
#26022=CARTESIAN_POINT ( 'NONE',  ( 37.29064029720369433, -289.1312849151976252, -256.0786889738105856 ) ) ;
#26023=CARTESIAN_POINT ( 'NONE',  ( -74.77521517568500542, -288.9132882718096198, -333.1661488197501058 ) ) ;
#26024=CARTESIAN_POINT ( 'NONE',  ( 18.31132212942786808, -286.3320889499269128, -217.1592540323484002 ) ) ;
#26026=CARTESIAN_POINT ( 'NONE',  ( -15.91953365755882999, -281.1702681912662456, -340.9835733159463302 ) ) ;
#26027=CARTESIAN_POINT ( 'NONE',  ( 35.77996097544042442, -289.2426465812927177, -257.2619838698184367 ) ) ;
#26028=CARTESIAN_POINT ( 'NONE',  ( -92.19394283087996200, -282.3341691312779176, -319.5933136778693324 ) ) ;
#26029=CARTESIAN_POINT ( 'NONE',  ( -103.8230523382779182, -280.2892044020557591, -238.9129695797552415 ) ) ;
#26030=CARTESIAN_POINT ( 'NONE',  ( -96.13880100621362601, -278.4369101236103461, -313.7513074768925208 ) ) ;
#26031=CARTESIAN_POINT ( 'NONE',  ( -111.6058214604120167, -289.5839374805772195, -251.5240505808429816 ) ) ;
#26032=CARTESIAN_POINT ( 'NONE',  ( -76.03426885895893861, -286.3522133154978633, -203.9142718908119321 ) ) ;
#26033=CARTESIAN_POINT ( 'NONE',  ( -67.17099252333942161, -286.1637426408757960, -199.4404565464750760 ) ) ;
#26034=CARTESIAN_POINT ( 'NONE',  ( 31.35531949319808476, -282.0494607849622639, -295.2030881855080224 ) ) ;
#26036=CARTESIAN_POINT ( 'NONE',  ( 144.7857639756989272, -299.5541904835127980, -201.0153591320744226 ) ) ;
#26037=CARTESIAN_POINT ( 'NONE',  ( -98.22635587058518070, -293.0220020018754781, -225.2465365023012112 ) ) ;
#26038=CARTESIAN_POINT ( 'NONE',  ( 21.83851085360088717, -291.5817081253803735, -221.8739969824914340 ) ) ;
#26039=CARTESIAN_POINT ( 'NONE',  ( 23.25373406459102199, -274.0405107072245414, -229.2095317962383092 ) ) ;
#26040=CARTESIAN_POINT ( 'NONE',  ( -113.8426565258949097, -295.8030002700830892, -278.1660175096241119 ) ) ;
#26041=CARTESIAN_POINT ( 'NONE',  ( -14.61435826916151370, -290.8320132361100718, -200.2599362279293302 ) ) ;
#26042=CARTESIAN_POINT ( 'NONE',  ( -26.07496108187088879, -293.1465899394908092, -343.5118842319939176 ) ) ;
#26043=CARTESIAN_POINT ( 'NONE',  ( -61.37059979273382737, -290.5764043571346633, -339.7134249763361140 ) ) ;
#26045=CARTESIAN_POINT ( 'NONE',  ( -59.41374184840418593, -291.3381026886466429, -342.0397453468048639 ) ) ;
#26046=CARTESIAN_POINT ( 'NONE',  ( 20.80757616961971479, -290.8968325258275058, -222.7303495992310047 ) ) ;
#26047=CARTESIAN_POINT ( 'NONE',  ( -23.05680853957240117, -296.8697261290107576, -344.0404940969793302 ) ) ;
#26048=CARTESIAN_POINT ( 'NONE',  ( -89.83986342218533139, -286.2300706523702729, -219.2261023316000887 ) ) ;
#26049=CARTESIAN_POINT ( 'NONE',  ( -14.31877491325872498, -296.7544549666146736, -341.9151069641986851 ) ) ;
#26050=CARTESIAN_POINT ( 'NONE',  ( 29.77367096495504839, -277.0811197690114795, -236.0984011776297109 ) ) ;
#26051=CARTESIAN_POINT ( 'NONE',  ( -71.40812745150046226, -276.2869881701229247, -338.9722486371768468 ) ) ;
#26052=CARTESIAN_POINT ( 'NONE',  ( -51.76026743750345815, -297.0694932703931386, -194.8332977247179372 ) ) ;
#26053=CARTESIAN_POINT ( 'NONE',  ( 36.71235791054292719, -273.8084387491682605, -271.6243233130498425 ) ) ;
#26054=CARTESIAN_POINT ( 'NONE',  ( -16.49548198456003689, -278.4034813065742355, -198.8995941773991945 ) ) ;
#26055=CARTESIAN_POINT ( 'NONE',  ( -91.42545596482558778, -274.4656484517480521, -220.7231790146008450 ) ) ;
#26056=CARTESIAN_POINT ( 'NONE',  ( 37.37310244894115385, -273.9243407237918291, -254.2896803181082248 ) ) ;
#26058=CARTESIAN_POINT ( 'NONE',  ( -37.15945358355362060, -298.8573334823564096, -197.1967596271784373 ) ) ;
#26059=DIRECTION ( 'NONE',  ( -1.000000000000000000, -0.000000000000000000, -0.000000000000000000 ) ) ;
#26060=CARTESIAN_POINT ( 'NONE',  ( -48.64766019395676722, -287.2153937429500274, -344.9161409946593153 ) ) ;
#26061=CARTESIAN_POINT ( 'NONE',  ( -27.28807909573529855, -274.0166624069921681, -198.0058300916056453 ) ) ;
#26063=CARTESIAN_POINT ( 'NONE',  ( -4.333064003954842036, -288.6290358601492585, -339.9416088546569767 ) ) ;
#26064=CARTESIAN_POINT ( 'NONE',  ( -97.27629017015085822, -289.5709119568793426, -318.6891446004945010 ) ) ;
#26065=CARTESIAN_POINT ( 'NONE',  ( -64.96310334541979614, -299.6731539603272836, -200.1949611922445058 ) ) ;
#26066=CARTESIAN_POINT ( 'NONE',  ( -37.01243542350478322, -293.0478298053715207, -345.2064670110290763 ) ) ;
#26068=CARTESIAN_POINT ( 'NONE',  ( 38.26484454770362476, -280.9219902866428811, -284.1384982832373680 ) ) ;
#26070=CIRCLE ( 'NONE', #48783, 3.038598599789554822 ) ;
#26071=CARTESIAN_POINT ( 'NONE',  ( -109.5054175807851493, -276.8170090409134900, -249.7470011854615279 ) ) ;
#26073=CARTESIAN_POINT ( 'NONE',  ( -18.38567190830197262, -287.5974808934334987, -341.3209646584199390 ) ) ;
#26075=CARTESIAN_POINT ( 'NONE',  ( -110.3691898909241473, -288.7721169183628831, -253.2175816028796476 ) ) ;
#26076=CARTESIAN_POINT ( 'NONE',  ( 13.96563049481983221, -276.3083346064670422, -217.4624830674252394 ) ) ;
#26077=CARTESIAN_POINT ( 'NONE',  ( -13.58774896038472590, -284.1749438286296368, -342.9858802593784617 ) ) ;
#26078=CARTESIAN_POINT ( 'NONE',  ( -56.93716887924511383, -295.8209000051339785, -197.5442296542422582 ) ) ;
#26079=CARTESIAN_POINT ( 'NONE',  ( -78.37662955577970081, -283.6216535731053909, -330.7360678116390886 ) ) ;
#26080=CARTESIAN_POINT ( 'NONE',  ( -34.03219620597342043, -275.5198675056001889, -196.8463432638048971 ) ) ;
#26081=CARTESIAN_POINT ( 'NONE',  ( 34.78312190811930549, -276.1924732490160750, -258.0143686126671696 ) ) ;
#26083=CARTESIAN_POINT ( 'NONE',  ( 35.26228161896224123, -283.7939573929965036, -289.1670342401912990 ) ) ;
#26084=CARTESIAN_POINT ( 'NONE',  ( -57.95958171669895620, -296.8379144666615161, -200.0879978985657033 ) ) ;
#26086=CARTESIAN_POINT ( 'NONE',  ( 203.5005663465542227, 292.0167436573144073, -53.99999999998427569 ) ) ;
#26087=CARTESIAN_POINT ( 'NONE',  ( 21.36627390962075879, -294.0570793758699892, -320.1845440882959224 ) ) ;
#26088=CARTESIAN_POINT ( 'NONE',  ( -97.09747876138567335, -287.1460866091586581, -225.6275318811606212 ) ) ;
#26090=CARTESIAN_POINT ( 'NONE',  ( -88.52914483777347243, -281.1952119285918457, -334.4957818155094174 ) ) ;
#26091=CARTESIAN_POINT ( 'NONE',  ( -101.9667318183248028, -277.2017182563430424, -312.0246084118936665 ) ) ;
#26092=CARTESIAN_POINT ( 'NONE',  ( -113.5898514270250814, -288.9414302369593770, -271.1994052677522404 ) ) ;
#26093=CARTESIAN_POINT ( 'NONE',  ( -93.94227847450628133, -285.4089046709201511, -317.5530906591745861 ) ) ;
#26094=CARTESIAN_POINT ( 'NONE',  ( -16.06846345869654513, -278.5335665624714352, -341.3050887445962758 ) ) ;
#26095=CARTESIAN_POINT ( 'NONE',  ( -34.48270525082197935, -284.4421412028659688, -346.7183864147860959 ) ) ;
#26096=CARTESIAN_POINT ( 'NONE',  ( -38.90886268173343865, -281.8671319001777533, -343.7540180332204045 ) ) ;
#26097=CARTESIAN_POINT ( 'NONE',  ( -66.88022731131943033, -281.6652702869935752, -201.4088982050968468 ) ) ;
#26098=CARTESIAN_POINT ( 'NONE',  ( -36.94186363751468605, -274.2237397348851573, -193.3491040225014501 ) ) ;
#26099=CARTESIAN_POINT ( 'NONE',  ( -98.80470547715859198, -277.7675484001170503, -316.7648563595901692 ) ) ;
#26100=CARTESIAN_POINT ( 'NONE',  ( -105.2402377331540038, -298.0677319908579079, -301.0010048126023321 ) ) ;
#26103=CARTESIAN_POINT ( 'NONE',  ( -102.7709606978420425, -295.1981239826878323, -232.0567677047278607 ) ) ;
#26104=CARTESIAN_POINT ( 'NONE',  ( 23.10676946594754355, -274.4893430611577969, -229.3024594146004915 ) ) ;
#26105=CARTESIAN_POINT ( 'NONE',  ( -106.4914070761503950, -274.1819324983832189, -237.4016467116934450 ) ) ;
#26106=CARTESIAN_POINT ( 'NONE',  ( 33.63545407948539179, -289.0379334093533998, -249.3350936155565876 ) ) ;
#26107=CARTESIAN_POINT ( 'NONE',  ( -96.85442100317582970, -297.4262955277986293, -318.1410186158751117 ) ) ;
#26108=CARTESIAN_POINT ( 'NONE',  ( 39.21063590991850845, -294.7922198035330439, -273.1447423540707860 ) ) ;
#26109=CARTESIAN_POINT ( 'NONE',  ( -97.22034534473348799, -291.9374302999586916, -315.2665251349304185 ) ) ;
#26110=CARTESIAN_POINT ( 'NONE',  ( 1.369612232640303517, -278.5700010460427052, -206.2584598251917498 ) ) ;
#26111=CARTESIAN_POINT ( 'NONE',  ( -88.53840235861714802, -281.2480841865800016, -216.2508744886622196 ) ) ;
#26112=CARTESIAN_POINT ( 'NONE',  ( -111.8143612772104944, -294.6537860262340587, -268.6763776530343080 ) ) ;
#26113=CARTESIAN_POINT ( 'NONE',  ( -37.29090667048291863, -284.9118958114838165, -346.1387607599690455 ) ) ;
#26114=CARTESIAN_POINT ( 'NONE',  ( 11.34959314314943235, -285.6659927943284742, -215.4897632967589800 ) ) ;
#26115=CARTESIAN_POINT ( 'NONE',  ( -102.4785513481026697, -256.8849682556987659, -326.4804194469078880 ) ) ;
#26117=CARTESIAN_POINT ( 'NONE',  ( -110.3303337026201660, -284.2476015338562547, -268.1823900040998296 ) ) ;
#26119=CARTESIAN_POINT ( 'NONE',  ( 24.33492938005380779, -282.0236205127432072, -224.7816721431527753 ) ) ;
#26121=CARTESIAN_POINT ( 'NONE',  ( -32.69392468982429278, -274.4455899300057240, -197.4755088537584982 ) ) ;
#26122=CARTESIAN_POINT ( 'NONE',  ( -43.61834939641957476, -284.7695806793934707, -193.9627842113003737 ) ) ;
#26123=CARTESIAN_POINT ( 'NONE',  ( -35.35417049297698355, -281.0177428821261287, -193.6090484366914950 ) ) ;
#26124=CARTESIAN_POINT ( 'NONE',  ( -77.14750778924423003, -281.0493906768019201, -205.1984387805477468 ) ) ;
#26125=CARTESIAN_POINT ( 'NONE',  ( -4.956745876385824090, -280.8002895305701827, -200.5258902693329617 ) ) ;
#26126=CARTESIAN_POINT ( 'NONE',  ( 34.45848030099739390, -285.0523547857347353, -270.3937649182068412 ) ) ;
#26127=CARTESIAN_POINT ( 'NONE',  ( -109.4453526793423066, -267.4301006796197271, -307.0599045550397364 ) ) ;
#26130=CARTESIAN_POINT ( 'NONE',  ( -77.57072815873762295, -275.5109923778701386, -207.2607714784864470 ) ) ;
#26131=CARTESIAN_POINT ( 'NONE',  ( 167.4490855713348481, 232.7245837427465176, -192.5400704262254976 ) ) ;
#26133=CARTESIAN_POINT ( 'NONE',  ( 34.53663548003434869, -279.8325073027585859, -290.4944653137752653 ) ) ;
#26134=CARTESIAN_POINT ( 'NONE',  ( 18.65356931988779721, -294.6040879910829062, -218.9947494755392370 ) ) ;
#26135=CARTESIAN_POINT ( 'NONE',  ( -95.69069826749094432, -295.2827579884799434, -314.4190790278208283 ) ) ;
#26136=CARTESIAN_POINT ( 'NONE',  ( -27.85045997660992256, -291.6771111854073411, -193.9566952136810301 ) ) ;
#26138=CARTESIAN_POINT ( 'NONE',  ( -108.8922377041888581, -294.7833688486718984, -297.3270354571271810 ) ) ;
#26139=CARTESIAN_POINT ( 'NONE',  ( 10.61987620586390335, -286.7767461549710220, -326.5190247029905777 ) ) ;
#26140=CARTESIAN_POINT ( 'NONE',  ( 35.28081334126409274, -295.6129955732050689, -285.8116592725950795 ) ) ;
#26141=CARTESIAN_POINT ( 'NONE',  ( -95.49646321174276409, -285.2386426385939444, -315.3179101848080563 ) ) ;
#26143=CARTESIAN_POINT ( 'NONE',  ( 30.69934612542391150, -294.9533403698755478, -305.9031527728337210 ) ) ;
#26145=CARTESIAN_POINT ( 'NONE',  ( -53.69735112532745802, -283.7599596137549156, -341.6205559743822278 ) ) ;
#26146=CARTESIAN_POINT ( 'NONE',  ( -86.15415973984993059, -294.5069593837021671, -329.3979920878251733 ) ) ;
#26147=CARTESIAN_POINT ( 'NONE',  ( -111.7630761765779539, -291.1145909481658691, -289.5348561627811250 ) ) ;
#26149=CARTESIAN_POINT ( 'NONE',  ( -111.1748761521547948, -291.3161115654262403, -248.7234420100204204 ) ) ;
#26150=CARTESIAN_POINT ( 'NONE',  ( 33.99555490870849184, -287.5144700297938130, -254.8693121371360917 ) ) ;
#26153=CARTESIAN_POINT ( 'NONE',  ( -107.7496587885240871, -298.7749155873104314, -242.2374380850581304 ) ) ;
#26155=CARTESIAN_POINT ( 'NONE',  ( -109.3808428249358542, -295.5642745168043461, -244.5995149352899887 ) ) ;
#26157=CARTESIAN_POINT ( 'NONE',  ( -57.16542497158069835, -278.8487626894216191, -199.8598528817571491 ) ) ;
#26159=CARTESIAN_POINT ( 'NONE',  ( -10.36331363604707789, -273.9024600337501170, -198.2510302314686328 ) ) ;
#26160=CARTESIAN_POINT ( 'NONE',  ( -86.54900706896299312, -295.8333841890787994, -215.5035871002841077 ) ) ;
#26161=CARTESIAN_POINT ( 'NONE',  ( -76.99593890458663736, -279.4495398642493456, -333.1782910029873506 ) ) ;
#26162=CARTESIAN_POINT ( 'NONE',  ( 33.24355366231290532, -273.3898002537761158, -247.2045609470798979 ) ) ;
#26163=CARTESIAN_POINT ( 'NONE',  ( 6.311353875102079236, -295.6497883543746639, -329.4290537440044773 ) ) ;
#26164=CARTESIAN_POINT ( 'NONE',  ( -71.82249880952453225, -298.6648180824919336, -205.6529596047545567 ) ) ;
#26166=CARTESIAN_POINT ( 'NONE',  ( -103.1690878561906004, -298.6581110149653568, -231.8748585589185893 ) ) ;
#26168=CARTESIAN_POINT ( 'NONE',  ( 17.73681752449018489, -296.7399187925757928, -195.2131683379656408 ) ) ;
#26169=CARTESIAN_POINT ( 'NONE',  ( -62.84405102379453467, -292.3625797558493105, -201.8518283426166420 ) ) ;
#26170=CARTESIAN_POINT ( 'NONE',  ( -110.2089398682156371, -288.9911257322809206, -280.7346875925552467 ) ) ;
#26172=CARTESIAN_POINT ( 'NONE',  ( 39.64587940594230275, -276.0545568708947144, -271.1647373776706900 ) ) ;
#26173=CARTESIAN_POINT ( 'NONE',  ( -69.49287347339856069, -273.7834252135151019, -204.8225640081446670 ) ) ;
#26174=CARTESIAN_POINT ( 'NONE',  ( -85.76743759011073109, -281.3659185024981753, -212.5578739362005933 ) ) ;
#26175=CARTESIAN_POINT ( 'NONE',  ( -21.84236188932190004, -281.5423374003972299, -345.2815343295065418 ) ) ;
#26177=CARTESIAN_POINT ( 'NONE',  ( -110.5721501603655952, -277.6033801587836365, -293.9977866416802499 ) ) ;
#26178=CARTESIAN_POINT ( 'NONE',  ( -109.3501439840259479, -283.9205375153651403, -257.3529300411557301 ) ) ;
#26179=CARTESIAN_POINT ( 'NONE',  ( 37.69716120803162340, -279.6185947863154979, -275.5600907017386589 ) ) ;
#26180=CARTESIAN_POINT ( 'NONE',  ( -69.73410430471044208, -272.1917306231412113, -204.2845936285694677 ) ) ;
#26181=CARTESIAN_POINT ( 'NONE',  ( -39.13295541706094838, -279.0747583980505624, -345.3523673384785866 ) ) ;
#26184=CARTESIAN_POINT ( 'NONE',  ( -54.34631544741656484, -296.0764771493508078, -196.3015671527024324 ) ) ;
#26185=CARTESIAN_POINT ( 'NONE',  ( -53.70668583079725522, -279.2617067182699202, -343.7780391190101454 ) ) ;
#26187=CARTESIAN_POINT ( 'NONE',  ( -101.6789132476428250, -285.9445193253832826, -309.9848129720878660 ) ) ;
#26190=CARTESIAN_POINT ( 'NONE',  ( 19.81465046686824394, -284.8797099097091632, -221.7807704580023653 ) ) ;
#26192=CARTESIAN_POINT ( 'NONE',  ( -66.22344206037546144, -294.2337965513641507, -337.8368579825529991 ) ) ;
#26193=CARTESIAN_POINT ( 'NONE',  ( -34.55497165967804563, -287.1564851326424446, -344.5944194559388052 ) ) ;
#26194=CARTESIAN_POINT ( 'NONE',  ( -78.59295187722810283, -208.2960365483323244, -357.4574221067172743 ) ) ;
#26195=CARTESIAN_POINT ( 'NONE',  ( -89.49879168472884317, -295.3175821871124072, -216.3939369506339006 ) ) ;
#26196=CARTESIAN_POINT ( 'NONE',  ( -29.51463500701300191, -284.6294643323478795, -194.4569362553195049 ) ) ;
#26197=CARTESIAN_POINT ( 'NONE',  ( 33.49683419924278382, -282.8814565027738013, -249.6646818075370220 ) ) ;
#26198=CARTESIAN_POINT ( 'NONE',  ( 10.20661578122992807, -278.9371163177303856, -211.0219832338596291 ) ) ;
#26199=CARTESIAN_POINT ( 'NONE',  ( -18.47350408722288861, -288.8023627039207213, -340.9331420923449514 ) ) ;
#26201=CARTESIAN_POINT ( 'NONE',  ( -91.74455907582854763, -280.6822924227491285, -220.8060591492271669 ) ) ;
#26202=CARTESIAN_POINT ( 'NONE',  ( -62.37378380844673131, -280.5209874317029062, -201.5617557106566835 ) ) ;
#26203=CARTESIAN_POINT ( 'NONE',  ( 22.53872477945380481, -288.9085317885618451, -224.5934783862951463 ) ) ;
#26207=CARTESIAN_POINT ( 'NONE',  ( -38.35741159830598690, -274.0397491378665791, -193.3678174284907243 ) ) ;
#26208=CARTESIAN_POINT ( 'NONE',  ( -76.71541153931548251, -291.5619509896136492, -333.7768703753266095 ) ) ;
#26210=CARTESIAN_POINT ( 'NONE',  ( 13.79469577742117714, -289.1948066931273615, -206.1857440867352693 ) ) ;
#26212=CARTESIAN_POINT ( 'NONE',  ( 13.62102484138827840, -274.3405803007165673, -325.6843491442355116 ) ) ;
#26214=CARTESIAN_POINT ( 'NONE',  ( -11.34944951100359134, -293.1190857903790743, -342.0469987695511236 ) ) ;
#26215=CARTESIAN_POINT ( 'NONE',  ( -35.80766856760973837, -297.5795176019383348, -197.2997115092137790 ) ) ;
#26217=CARTESIAN_POINT ( 'NONE',  ( 24.09814257179160180, -289.6318585424685921, -311.0763553971066244 ) ) ;
#26219=CARTESIAN_POINT ( 'NONE',  ( -13.17763998383056112, -284.4941976333578282, -340.3731186695097222 ) ) ;
#26220=CARTESIAN_POINT ( 'NONE',  ( -86.15070591020423763, -292.8161348075420847, -211.5022055586851195 ) ) ;
#26221=CARTESIAN_POINT ( 'NONE',  ( -101.8762173958342032, -291.3240794711874742, -311.5510866003369301 ) ) ;
#26222=CARTESIAN_POINT ( 'NONE',  ( -4.957521955928856805, -288.4785857780137235, -202.6988564975496558 ) ) ;
#26223=CARTESIAN_POINT ( 'NONE',  ( -95.90718960166142892, -279.3932942819733398, -220.3500321010474465 ) ) ;
#26224=CARTESIAN_POINT ( 'NONE',  ( -107.5415120038456820, -294.9949542721644207, -242.2688745684934304 ) ) ;
#26225=CARTESIAN_POINT ( 'NONE',  ( -30.21700538607526454, -282.7976833110919301, -347.0307907961067144 ) ) ;
#26226=AXIS2_PLACEMENT_3D ( 'NONE', #59272, #37923, #67312 ) ;
#26227=CARTESIAN_POINT ( 'NONE',  ( 32.26848328570245883, -277.0743390925360359, -244.5679436159495879 ) ) ;
#26228=CARTESIAN_POINT ( 'NONE',  ( -6.998514795304313196, -276.9805209788415823, -207.2794874003663779 ) ) ;
#26229=CARTESIAN_POINT ( 'NONE',  ( -71.04305100123842465, -275.6317540362420004, -338.2177641835416466 ) ) ;
#26231=CARTESIAN_POINT ( 'NONE',  ( 25.19220096963838529, -280.5390123121077863, -232.4807961771055886 ) ) ;
#26233=CARTESIAN_POINT ( 'NONE',  ( -104.6194925268544296, -279.2807441141486606, -306.9904418572131135 ) ) ;
#26234=CARTESIAN_POINT ( 'NONE',  ( -70.95236317204168586, -284.6782047952333414, -201.3455868035404137 ) ) ;
#26235=CARTESIAN_POINT ( 'NONE',  ( 24.17114297115016086, -294.7484841682050387, -229.2011356279915333 ) ) ;
#26236=CARTESIAN_POINT ( 'NONE',  ( 37.94857302815160693, -277.3048287523072872, -282.4323135914204386 ) ) ;
#26237=CARTESIAN_POINT ( 'NONE',  ( 0.9341010739579499456, -275.8668556970181953, -204.1019794387270849 ) ) ;
#26239=CARTESIAN_POINT ( 'NONE',  ( 35.58709516685505037, -275.3298018247866139, -266.1410867121336423 ) ) ;
#26240=CARTESIAN_POINT ( 'NONE',  ( -111.0867660119768061, -298.7159470455799806, -257.6452347675588044 ) ) ;
#26241=CARTESIAN_POINT ( 'NONE',  ( -38.63158897254069046, -284.0358156053305834, -195.5261024270406836 ) ) ;
#26242=CARTESIAN_POINT ( 'NONE',  ( 34.44464787985057086, -292.8650257537631774, -242.4205436915711687 ) ) ;
#26243=CARTESIAN_POINT ( 'NONE',  ( 37.50056638392412367, -288.9712979445082510, -256.0406584779146897 ) ) ;
#26245=CARTESIAN_POINT ( 'NONE',  ( 34.62521702829261727, -292.6559072008711269, -284.3249609128792486 ) ) ;
#26247=CARTESIAN_POINT ( 'NONE',  ( 12.90476180693938879, -291.3124891340683575, -212.7946402857659223 ) ) ;
#26248=CARTESIAN_POINT ( 'NONE',  ( 23.36118198553759839, -292.6553995129997929, -229.7748199266951588 ) ) ;
#26250=CARTESIAN_POINT ( 'NONE',  ( 38.37206299093478634, -288.7891116113618182, -282.8875521945520859 ) ) ;
#26251=CARTESIAN_POINT ( 'NONE',  ( -76.83686048527216883, -279.8408640855582803, -208.8824401048894686 ) ) ;
#26252=CARTESIAN_POINT ( 'NONE',  ( -56.00840384629794499, -294.2074439675961912, -344.7455698604939016 ) ) ;
#26253=CARTESIAN_POINT ( 'NONE',  ( -60.48715447031707981, -286.4111992367593302, -196.9734871406977277 ) ) ;
#26254=CARTESIAN_POINT ( 'NONE',  ( -35.15309205289024419, -286.4121743407843041, -193.4002407481139301 ) ) ;
#26255=CARTESIAN_POINT ( 'NONE',  ( -42.93030043953837094, -283.4577701810317194, -343.2181901583103354 ) ) ;
#26256=CARTESIAN_POINT ( 'NONE',  ( 203.1404359220460094, 295.9636561932003929, -68.66402283083226621 ) ) ;
#26257=CARTESIAN_POINT ( 'NONE',  ( -85.03340929734007148, -218.4748483833227510, -351.2754620631345119 ) ) ;
#26258=CARTESIAN_POINT ( 'NONE',  ( 120.5147935217607369, 148.1047250371406108, -260.3425545554943028 ) ) ;
#26259=CARTESIAN_POINT ( 'NONE',  ( 31.27329421153728006, -274.4115196545928370, -244.9724536127689589 ) ) ;
#26260=CARTESIAN_POINT ( 'NONE',  ( -39.17923399095218429, -275.9960779647041704, -343.6471981327445633 ) ) ;
#26261=CARTESIAN_POINT ( 'NONE',  ( -113.5925088572683421, -295.9264570160129892, -281.0151233285136527 ) ) ;
#26262=CARTESIAN_POINT ( 'NONE',  ( -110.3569200167271731, -272.2263580403405285, -270.3569698429222399 ) ) ;
#26263=CARTESIAN_POINT ( 'NONE',  ( 21.34152340402464887, -274.9018619669350869, -319.4485659730281100 ) ) ;
#26264=CARTESIAN_POINT ( 'NONE',  ( -95.42165565302137509, -274.9507823595713489, -224.4841871472521291 ) ) ;
#26266=CARTESIAN_POINT ( 'NONE',  ( -36.91058164494567961, -298.9986726998774884, -193.5963432578485310 ) ) ;
#26267=CARTESIAN_POINT ( 'NONE',  ( 31.89691442077901584, -287.7349170331864343, -247.0372525869651383 ) ) ;
#26268=CARTESIAN_POINT ( 'NONE',  ( -44.76981581364312035, -295.9465974294657826, -346.8930492274545827 ) ) ;
#26269=CARTESIAN_POINT ( 'NONE',  ( -93.62202212357776432, -297.7608938521111099, -217.8233932158630637 ) ) ;
#26270=CARTESIAN_POINT ( 'NONE',  ( 18.83445677758343351, -294.3800209773427241, -316.9791338116584143 ) ) ;
#26272=CARTESIAN_POINT ( 'NONE',  ( 13.92446225311632446, -278.2602636349503769, -325.9399616888951527 ) ) ;
#26274=CARTESIAN_POINT ( 'NONE',  ( 20.08693444838612407, -280.3649296713189187, -219.1409270331742221 ) ) ;
#26276=CARTESIAN_POINT ( 'NONE',  ( 21.03170101262399072, -277.1128943885149170, -314.5872922240578191 ) ) ;
#26277=CARTESIAN_POINT ( 'NONE',  ( -9.561140581058900523, -278.4542155220726727, -341.0874534253259185 ) ) ;
#26278=CARTESIAN_POINT ( 'NONE',  ( -111.3753964750786167, -276.7527005194771164, -256.2416556145506092 ) ) ;
#26279=CARTESIAN_POINT ( 'NONE',  ( -60.55611930151117406, -298.3944916406449011, -200.9895843317770243 ) ) ;
#26280=CARTESIAN_POINT ( 'NONE',  ( -55.96985377278768681, -293.8713545529170688, -341.6063911346960822 ) ) ;
#26282=CARTESIAN_POINT ( 'NONE',  ( 23.69465426782590711, -281.4189287664364088, -223.4984796440012360 ) ) ;
#26283=CARTESIAN_POINT ( 'NONE',  ( -110.2800522210475691, -278.6792653490147700, -273.3605843429757556 ) ) ;
#26285=CARTESIAN_POINT ( 'NONE',  ( 33.57885181016307286, -286.6052818202414301, -299.2001241953170734 ) ) ;
#26286=CARTESIAN_POINT ( 'NONE',  ( -86.73877593368048622, -275.3659278562917052, -213.8568694637461647 ) ) ;
#26288=CIRCLE ( 'NONE', #15757, 2.500000000000008882 ) ;
#26289=CARTESIAN_POINT ( 'NONE',  ( -84.79752433890394059, -288.9230149066366380, -326.1105451711822525 ) ) ;
#26290=VECTOR ( 'NONE', #50479, 999.9999999999998863 ) ;
#26291=CARTESIAN_POINT ( 'NONE',  ( -88.26026055514134327, -283.0916473165418097, -328.0569839667695646 ) ) ;
#26292=CARTESIAN_POINT ( 'NONE',  ( 35.21975468809848309, -279.9826426000877859, -285.0127886254265945 ) ) ;
#26293=CARTESIAN_POINT ( 'NONE',  ( 32.54184616499231453, -279.8213389707801184, -247.1425293020669187 ) ) ;
#26294=CARTESIAN_POINT ( 'NONE',  ( -59.39767046211024137, -281.4196310038104230, -341.5127707078032699 ) ) ;
#26295=CARTESIAN_POINT ( 'NONE',  ( -55.21721882969501394, -287.8225279027227543, -197.4696047219434547 ) ) ;
#26296=CARTESIAN_POINT ( 'NONE',  ( -108.6792038926475641, -279.9837929090616626, -253.0958041212535932 ) ) ;
#26298=CARTESIAN_POINT ( 'NONE',  ( 20.64628258383619297, -294.8965061006154542, -222.7964828649481603 ) ) ;
#26300=CARTESIAN_POINT ( 'NONE',  ( -68.61902918569309406, -275.6974156703191738, -339.6263475907481961 ) ) ;
#26301=CARTESIAN_POINT ( 'NONE',  ( 32.99820258467713785, -276.4668849976455931, -290.3114866442770108 ) ) ;
#26302=CARTESIAN_POINT ( 'NONE',  ( -110.0939359457274520, -286.3094202302920053, -289.3102426970918941 ) ) ;
#26304=CARTESIAN_POINT ( 'NONE',  ( -108.5010049489971351, -292.1436745756881237, -295.9260817014101121 ) ) ;
#26305=CARTESIAN_POINT ( 'NONE',  ( -101.4931958176359359, -294.0302014091283809, -309.3126913038948373 ) ) ;
#26308=CARTESIAN_POINT ( 'NONE',  ( 34.86110644327963826, -274.0573143454735714, -256.6498743373807088 ) ) ;
#26309=CARTESIAN_POINT ( 'NONE',  ( -28.77659480126357749, -293.0821270705926054, -344.1524296968357817 ) ) ;
#26312=CARTESIAN_POINT ( 'NONE',  ( -61.45100030471474639, -290.2245802948023083, -197.9076169380507224 ) ) ;
#26313=CARTESIAN_POINT ( 'NONE',  ( -81.97845966521933292, -287.0321949051790966, -211.5903760177906747 ) ) ;
#26314=CARTESIAN_POINT ( 'NONE',  ( -79.99064857901045400, -287.8600200346054407, -333.3138133357191464 ) ) ;
#26315=CARTESIAN_POINT ( 'NONE',  ( -52.22570088316209080, -287.2831139814683752, -198.2928070756119610 ) ) ;
#26317=CARTESIAN_POINT ( 'NONE',  ( -95.90131998200267560, -285.9692173225861893, -226.5048453415226675 ) ) ;
#26318=CARTESIAN_POINT ( 'NONE',  ( 0.8443782721789957479, -294.5383403931590465, -205.3381969002995788 ) ) ;
#26319=CARTESIAN_POINT ( 'NONE',  ( 37.07818616452597382, -273.4644007121743812, -257.2105570007907431 ) ) ;
#26320=CARTESIAN_POINT ( 'NONE',  ( 30.52642916392602856, -276.3563393324366189, -306.8008231461516289 ) ) ;
#26321=CARTESIAN_POINT ( 'NONE',  ( -28.00236521333965811, -290.2495343561877235, -195.3278414869026278 ) ) ;
#26322=CARTESIAN_POINT ( 'NONE',  ( -71.23459404651939053, -279.6170165848312195, -201.2216087144612402 ) ) ;
#26323=CARTESIAN_POINT ( 'NONE',  ( -67.94705255485008877, -297.4357834180092937, -338.4571338914789749 ) ) ;
#26326=CARTESIAN_POINT ( 'NONE',  ( -62.71753342243975737, -284.3997853769526500, -201.3335911245622754 ) ) ;
#26327=CARTESIAN_POINT ( 'NONE',  ( -110.2609925786772749, -276.5103471030346327, -284.3439342227755446 ) ) ;
#26329=CARTESIAN_POINT ( 'NONE',  ( 37.53077405354408569, -279.6185947847861826, -275.5486191957865003 ) ) ;
#26332=CARTESIAN_POINT ( 'NONE',  ( 22.22934109539131597, -273.3872836693557815, -222.6539268636627469 ) ) ;
#26333=CARTESIAN_POINT ( 'NONE',  ( -110.0062987976195075, -277.7896554108201599, -278.7933480222311573 ) ) ;
#26334=CARTESIAN_POINT ( 'NONE',  ( 14.82059547345917316, -295.8212091062537183, -322.4886528285321106 ) ) ;
#26335=CARTESIAN_POINT ( 'NONE',  ( -39.56446820536647380, -278.9452208197390632, -193.6894486889392226 ) ) ;
#26336=CARTESIAN_POINT ( 'NONE',  ( -96.59173980530474068, -296.8926654562826002, -313.4271606224881452 ) ) ;
#26337=CARTESIAN_POINT ( 'NONE',  ( -84.92288838259740658, -298.7263989168827152, -210.4501106825119336 ) ) ;
#26338=CARTESIAN_POINT ( 'NONE',  ( -52.63301758662038310, -297.6842090015859412, -198.9287340268444950 ) ) ;
#26339=CARTESIAN_POINT ( 'NONE',  ( -44.51620921233904227, -293.9616707821442105, -195.6528484282623310 ) ) ;
#26340=CARTESIAN_POINT ( 'NONE',  ( -15.41548952005958206, -286.4948914133883591, -196.4935233328399136 ) ) ;
#26341=CARTESIAN_POINT ( 'NONE',  ( 36.43760177122948107, -273.4720743667242004, -253.0732350519316469 ) ) ;
#26342=CARTESIAN_POINT ( 'NONE',  ( 5.555563528388226757, -288.3217801799153790, -334.3050369684871725 ) ) ;
#26343=CARTESIAN_POINT ( 'NONE',  ( -65.45853539776376806, -281.6626226006118827, -201.2142425780098165 ) ) ;
#26344=CARTESIAN_POINT ( 'NONE',  ( -0.8846859871772232431, -287.6144534260129717, -333.9355825978587973 ) ) ;
#26345=CARTESIAN_POINT ( 'NONE',  ( -95.88598520365640354, -289.1967194205273586, -223.4828998136632663 ) ) ;
#26347=CARTESIAN_POINT ( 'NONE',  ( -75.88346903603265048, -208.4961600436150491, -353.2410745688453062 ) ) ;
#26349=CARTESIAN_POINT ( 'NONE',  ( -71.20684811354948351, -289.0195022834400902, -335.1142689583439847 ) ) ;
#26351=CARTESIAN_POINT ( 'NONE',  ( -47.21419329412872656, -284.1159239877375740, -346.4883410451242867 ) ) ;
#26352=CARTESIAN_POINT ( 'NONE',  ( -90.61399526793843506, -290.3784373443359073, -215.0163613484924952 ) ) ;
#26353=CARTESIAN_POINT ( 'NONE',  ( 30.00512399797122498, -282.6858058148495161, -234.5997591034260665 ) ) ;
#26354=CARTESIAN_POINT ( 'NONE',  ( 21.58012721499826370, -282.2070399355927748, -221.5603337975484237 ) ) ;
#26355=CARTESIAN_POINT ( 'NONE',  ( 31.97727590711572887, -281.0797282946595033, -247.3133679471492599 ) ) ;
#26356=CARTESIAN_POINT ( 'NONE',  ( -4.453409786974630968, -276.4856637636619894, -202.9424595835075138 ) ) ;
#26357=CARTESIAN_POINT ( 'NONE',  ( -86.39531758579973086, -295.7118411637598001, -329.7138147562689028 ) ) ;
#26359=CARTESIAN_POINT ( 'NONE',  ( -108.9665960450441133, -288.8447249982889389, -249.2986243628762395 ) ) ;
#26360=CARTESIAN_POINT ( 'NONE',  ( -110.7387727487133446, -271.3472703583528869, -270.3458102218887120 ) ) ;
#26363=CARTESIAN_POINT ( 'NONE',  ( -89.89389982017860348, -285.7208645413335262, -323.1551704498491517 ) ) ;
#26365=CARTESIAN_POINT ( 'NONE',  ( -68.08957639106087356, -296.5262102990658946, -340.6182216507805833 ) ) ;
#26367=CARTESIAN_POINT ( 'NONE',  ( 11.99158077817589607, -282.9956912279861285, -324.3066466475954144 ) ) ;
#26368=CARTESIAN_POINT ( 'NONE',  ( 35.83470535471820284, -274.9033446749280074, -293.5566756073033616 ) ) ;
#26369=CARTESIAN_POINT ( 'NONE',  ( -96.50576685131620991, -291.8651355981500046, -221.2192231310186799 ) ) ;
#26370=CARTESIAN_POINT ( 'NONE',  ( -75.46437946928794815, -283.6893944842710766, -204.8257800826843891 ) ) ;
#26371=CARTESIAN_POINT ( 'NONE',  ( 6.480709740987499856, -292.9632695087938714, -207.0733570431969497 ) ) ;
#26372=CARTESIAN_POINT ( 'NONE',  ( -53.40905182814710628, -289.5972684268609214, -341.5926257303513580 ) ) ;
#26376=CARTESIAN_POINT ( 'NONE',  ( 201.4066894621335280, 289.8166775212674224, -82.35935531522035546 ) ) ;
#26377=CARTESIAN_POINT ( 'NONE',  ( -55.51810208605158437, -284.8020765033892303, -344.4713477943891462 ) ) ;
#26378=CARTESIAN_POINT ( 'NONE',  ( 35.78497577281001440, -278.8380690714489560, -253.7030783399848985 ) ) ;
#26380=CARTESIAN_POINT ( 'NONE',  ( 34.06459102718468301, -280.2544932693967894, -253.7669124225878647 ) ) ;
#26381=CARTESIAN_POINT ( 'NONE',  ( -6.587047800884924698, -276.3259785197055862, -340.9437455100886041 ) ) ;
#26382=CARTESIAN_POINT ( 'NONE',  ( -8.565318823985945684, -282.4298136066522602, -201.2818279806009230 ) ) ;
#26383=CARTESIAN_POINT ( 'NONE',  ( 7.652886109949530002, -59.88684688645761156, -352.9270608465728856 ) ) ;
#26384=CARTESIAN_POINT ( 'NONE',  ( -3.898980447687987461, -279.0593657860032408, -201.6430641607024938 ) ) ;
#26385=CARTESIAN_POINT ( 'NONE',  ( -97.89467229529081749, -283.1694792728249013, -226.6909045270137995 ) ) ;
#26386=CARTESIAN_POINT ( 'NONE',  ( -43.23384418626412184, -299.7389936128457180, -194.5507258692761354 ) ) ;
#26388=CARTESIAN_POINT ( 'NONE',  ( 34.12908445250047151, -294.2451482167011250, -285.5841125330833847 ) ) ;
#26390=CARTESIAN_POINT ( 'NONE',  ( -106.1666134912603070, -289.5802534498914156, -244.4413347145414264 ) ) ;
#26391=CARTESIAN_POINT ( 'NONE',  ( 29.01218391079727255, -276.7101048117015125, -309.2259460319469895 ) ) ;
#26392=CARTESIAN_POINT ( 'NONE',  ( 20.68153027937933430, -274.9289478228903363, -226.0426334068589540 ) ) ;
#26393=CARTESIAN_POINT ( 'NONE',  ( 36.93591799251217367, -274.7123195487147314, -289.4484948865908791 ) ) ;
#26395=CARTESIAN_POINT ( 'NONE',  ( -109.9060790237128344, -270.7979523233628925, -251.2056178072172941 ) ) ;
#26398=CARTESIAN_POINT ( 'NONE',  ( 18.73967121504439604, -283.2998504914871774, -317.5940168848536018 ) ) ;
#26399=CARTESIAN_POINT ( 'NONE',  ( 34.65625571128948224, -283.6242464919540112, -294.8202209381691432 ) ) ;
#26400=CARTESIAN_POINT ( 'NONE',  ( -110.1980361825345653, -283.8218637189545461, -276.3483514582993621 ) ) ;
#26401=CARTESIAN_POINT ( 'NONE',  ( 25.97253327641737997, -273.4349648419598680, -232.3444398746385389 ) ) ;
#26402=CARTESIAN_POINT ( 'NONE',  ( 17.96755236496446173, -282.7158978469478257, -220.8459478810472660 ) ) ;
#26403=CARTESIAN_POINT ( 'NONE',  ( 27.36637378483180782, -274.5101507844141224, -305.7320739244359515 ) ) ;
#26405=CARTESIAN_POINT ( 'NONE',  ( 11.74333479298099014, -275.8322769167834281, -215.8420162428405717 ) ) ;
#26407=CARTESIAN_POINT ( 'NONE',  ( -73.69828186844009110, -280.3849564428605277, -202.6530829540375009 ) ) ;
#26409=FACE_OUTER_BOUND ( 'NONE', #3280, .T. ) ;
#26410=CARTESIAN_POINT ( 'NONE',  ( -73.05211475263534737, -287.4448424621183449, -203.4818108167443427 ) ) ;
#26411=CARTESIAN_POINT ( 'NONE',  ( -63.63655701532286457, -294.6009067051807619, -338.6876494883055102 ) ) ;
#26412=CARTESIAN_POINT ( 'NONE',  ( -113.7133381119638074, -289.7827442907640147, -279.7835390527013715 ) ) ;
#26413=CARTESIAN_POINT ( 'NONE',  ( 36.28469113919991429, -285.6936628434098111, -262.8027768066472163 ) ) ;
#26414=CARTESIAN_POINT ( 'NONE',  ( 33.60210927526537006, -285.8705693364300942, -250.8073248591778395 ) ) ;
#26415=CARTESIAN_POINT ( 'NONE',  ( -109.6965320845570346, -288.9947285975260911, -254.7806074367004499 ) ) ;
#26416=CARTESIAN_POINT ( 'NONE',  ( -106.5429952969378036, -285.4316695667433805, -294.9727740246291319 ) ) ;
#26417=CARTESIAN_POINT ( 'NONE',  ( -17.90150196408593430, -274.8013122873251177, -342.7978444491726577 ) ) ;
#26418=CARTESIAN_POINT ( 'NONE',  ( -49.19991959951759952, -284.3034606604090868, -195.0362803112939787 ) ) ;
#26419=CARTESIAN_POINT ( 'NONE',  ( -99.89601474075350040, -299.1113143508848111, -228.9619021200954876 ) ) ;
#26420=CARTESIAN_POINT ( 'NONE',  ( 10.92043478843026172, -284.7174067739193219, -212.6668424218146924 ) ) ;
#26421=CARTESIAN_POINT ( 'NONE',  ( 19.00949645153776046, -281.8319373625953403, -223.5661195490816908 ) ) ;
#26422=CARTESIAN_POINT ( 'NONE',  ( -59.46284473111802527, -291.3381026873716451, -342.1990145676941779 ) ) ;
#26425=CARTESIAN_POINT ( 'NONE',  ( -22.35871999816993494, -296.7818865975477252, -344.4207189917935921 ) ) ;
#26426=CARTESIAN_POINT ( 'NONE',  ( -109.1344211384381566, -276.8316147073302886, -248.6630567903306144 ) ) ;
#26427=CARTESIAN_POINT ( 'NONE',  ( -0.8714687899061585030, -291.7210559669639451, -202.7291651278841300 ) ) ;
#26428=CARTESIAN_POINT ( 'NONE',  ( -109.3771439809073627, -294.7427000464688263, -286.4027901715789994 ) ) ;
#26429=CARTESIAN_POINT ( 'NONE',  ( 10.21514642313670329, -281.0652302525782602, -326.4600721717990837 ) ) ;
#26430=CARTESIAN_POINT ( 'NONE',  ( 22.65603105917831073, -273.0266130720748379, -226.2976812982627735 ) ) ;
#26431=CARTESIAN_POINT ( 'NONE',  ( 34.69657940652931671, -294.6766661292332401, -255.8101812088421241 ) ) ;
#26432=CARTESIAN_POINT ( 'NONE',  ( -37.30987171927208124, -297.5519495502701943, -345.3611179825600175 ) ) ;
#26433=CARTESIAN_POINT ( 'NONE',  ( -113.6731869624870939, -295.0059029413213239, -272.4314892816096858 ) ) ;
#26435=CARTESIAN_POINT ( 'NONE',  ( 22.36139224206100096, -292.4292534763379763, -317.3874628399476592 ) ) ;
#26436=CARTESIAN_POINT ( 'NONE',  ( -100.8029659881560889, -291.4687410338707423, -307.7178867496866701 ) ) ;
#26439=CARTESIAN_POINT ( 'NONE',  ( -103.7070790576606214, -291.7697287510218302, -239.5676413039495571 ) ) ;
#26441=CARTESIAN_POINT ( 'NONE',  ( 3.629792614694514086, -280.5244457648807384, -333.6663039421703729 ) ) ;
#26442=CARTESIAN_POINT ( 'NONE',  ( 26.23455502610557843, -293.0598504924863619, -234.3822895747496773 ) ) ;
#26443=CARTESIAN_POINT ( 'NONE',  ( 8.546538727886705544, -280.6610364103018469, -208.4622460652895484 ) ) ;
#26444=CARTESIAN_POINT ( 'NONE',  ( -70.46486825586555369, -283.1435913071669574, -339.8637045638298559 ) ) ;
#26445=CARTESIAN_POINT ( 'NONE',  ( -56.56040196355512251, -287.3001343400755445, -342.7383702791111091 ) ) ;
#26446=CARTESIAN_POINT ( 'NONE',  ( -108.1713766829209789, -282.4020454386303527, -292.5877326523000193 ) ) ;
#26447=ADVANCED_FACE ( 'NONE', ( #15595 ), #70094, .T. ) ;
#26448=CARTESIAN_POINT ( 'NONE',  ( -67.07429098632485420, -278.1492807548430619, -200.0853697151221695 ) ) ;
#26449=AXIS2_PLACEMENT_3D ( 'NONE', #73417, #30315, #88051 ) ;
#26450=CARTESIAN_POINT ( 'NONE',  ( 36.39783940363580683, -286.2051470655875960, -249.1017686944038587 ) ) ;
#26452=CARTESIAN_POINT ( 'NONE',  ( 36.44263436832511616, -295.1932846108848025, -273.5029255886173587 ) ) ;
#26453=CARTESIAN_POINT ( 'NONE',  ( -37.11038484630563516, -278.4745399033110402, -346.7845003415363294 ) ) ;
#26454=CARTESIAN_POINT ( 'NONE',  ( -109.9866872626672887, -278.3228762974750907, -262.4745185282186526 ) ) ;
#26455=CARTESIAN_POINT ( 'NONE',  ( -99.20585895683687738, -291.3285398980592049, -224.4933552157917234 ) ) ;
#26456=CARTESIAN_POINT ( 'NONE',  ( -94.26629997111695047, -281.9472363966891635, -320.0491862950931932 ) ) ;
#26457=CARTESIAN_POINT ( 'NONE',  ( 13.07378857589137766, -291.8365520526449473, -217.2415646481958049 ) ) ;
#26458=CARTESIAN_POINT ( 'NONE',  ( -110.9214670853182980, -294.7393583532002026, -255.7687070272976939 ) ) ;
#26461=CARTESIAN_POINT ( 'NONE',  ( -6.744843068460973257, -294.1469356056429092, -336.7073370152170924 ) ) ;
#26463=CARTESIAN_POINT ( 'NONE',  ( 7.450504543161054372, -284.1952119285919025, -214.2458315076590907 ) ) ;
#26464=CARTESIAN_POINT ( 'NONE',  ( -73.16013433214311590, -296.6482473316476671, -202.4065082351918647 ) ) ;
#26465=CARTESIAN_POINT ( 'NONE',  ( 35.00342103530817184, -279.4044136373784113, -247.8558091756340218 ) ) ;
#26466=CARTESIAN_POINT ( 'NONE',  ( -60.37749554774559613, -287.0748531455805619, -197.3493967724697313 ) ) ;
#26467=CARTESIAN_POINT ( 'NONE',  ( -71.17464494521304630, -289.3451167832467945, -335.0616523255988568 ) ) ;
#26468=CARTESIAN_POINT ( 'NONE',  ( -110.5909649590966382, -279.9608405907517295, -278.8890940655768986 ) ) ;
#26469=CARTESIAN_POINT ( 'NONE',  ( -97.75412229689837318, -293.9719932934322628, -314.2256865053174693 ) ) ;
#26470=CARTESIAN_POINT ( 'NONE',  ( -101.0271346666929162, -297.7999964378646496, -308.1732457859682199 ) ) ;
#26471=CARTESIAN_POINT ( 'NONE',  ( -110.3594849809585696, -277.4512222227780853, -262.4229063633192709 ) ) ;
#26473=CARTESIAN_POINT ( 'NONE',  ( 19.37362162970248747, -298.4107710989599127, -193.3853472190476737 ) ) ;
#26474=CARTESIAN_POINT ( 'NONE',  ( -111.1308226261956236, -292.6043353087607102, -260.1554553659917133 ) ) ;
#26475=CARTESIAN_POINT ( 'NONE',  ( 30.20273208727713055, -295.6121107140541540, -305.6341968131068256 ) ) ;
#26476=CARTESIAN_POINT ( 'NONE',  ( -113.9037752538512365, -273.8091386319557046, -270.3771224311939818 ) ) ;
#26477=CARTESIAN_POINT ( 'NONE',  ( 12.23100940161551087, -288.9919839168108524, -324.1555013309709352 ) ) ;
#26479=CARTESIAN_POINT ( 'NONE',  ( -93.59385938653188930, -297.9199342052745578, -217.8524608410955352 ) ) ;
#26480=CARTESIAN_POINT ( 'NONE',  ( -96.48426051456434038, -289.3364413222395797, -223.0064662996730931 ) ) ;
#26481=CARTESIAN_POINT ( 'NONE',  ( -37.25787227667515111, -298.3864558371908515, -193.3814936317900504 ) ) ;
#26485=CARTESIAN_POINT ( 'NONE',  ( -71.57788828196257214, -291.0163332232990001, -338.5563610408362933 ) ) ;
#26486=CARTESIAN_POINT ( 'NONE',  ( 36.60358173371528068, -284.4805209788416391, -305.9350535429201159 ) ) ;
#26487=CARTESIAN_POINT ( 'NONE',  ( -4.979328192849334478, -279.8157544748613645, -200.6044719207231992 ) ) ;
#26488=CARTESIAN_POINT ( 'NONE',  ( -94.67573691093001287, -287.2184767517394448, -222.2691575733643390 ) ) ;
#26489=CARTESIAN_POINT ( 'NONE',  ( 37.71483743257300603, -285.9463863177180656, -256.0390209431961352 ) ) ;
#26490=CARTESIAN_POINT ( 'NONE',  ( 35.62697380994278262, -273.3376967091575125, -253.7025017441659145 ) ) ;
#26491=CARTESIAN_POINT ( 'NONE',  ( -68.91516944485796614, -275.5539532124696507, -202.9347589601644302 ) ) ;
#26492=CARTESIAN_POINT ( 'NONE',  ( -109.1207670723014900, -288.3741955690873056, -290.2764115782188128 ) ) ;
#26493=CARTESIAN_POINT ( 'NONE',  ( -90.44610022641995783, -279.6543113907909515, -324.4736994991283723 ) ) ;
#26495=CARTESIAN_POINT ( 'NONE',  ( 22.11349279239495047, -280.9604616252137248, -228.0045360289964833 ) ) ;
#26496=CARTESIAN_POINT ( 'NONE',  ( 35.78954898484706604, -280.8773950475191441, -268.5893716310541777 ) ) ;
#26497=CARTESIAN_POINT ( 'NONE',  ( 36.94277344190060575, -276.8713131571805661, -289.4217973297370463 ) ) ;
#26498=CARTESIAN_POINT ( 'NONE',  ( 21.67465908354142101, -279.6871979201942509, -221.5238569468187961 ) ) ;
#26499=CARTESIAN_POINT ( 'NONE',  ( -32.16148137795721595, -124.0225950033424880, -361.1636328524395481 ) ) ;
#26500=CARTESIAN_POINT ( 'NONE',  ( 39.14707202085495652, -276.5749793860932186, -276.8640363753513611 ) ) ;
#26501=CARTESIAN_POINT ( 'NONE',  ( -23.51092029594954269, -299.6473766074118998, -193.9470657638637192 ) ) ;
#26502=CARTESIAN_POINT ( 'NONE',  ( 21.31550574532285580, -290.6948066931273615, -317.0979686699210447 ) ) ;
#26505=CARTESIAN_POINT ( 'NONE',  ( 32.61271130941165097, -288.9231535424723916, -292.4529101380038583 ) ) ;
#26506=CARTESIAN_POINT ( 'NONE',  ( 21.63305556083389902, -289.9638667322107040, -318.2976992908221519 ) ) ;
#26507=CARTESIAN_POINT ( 'NONE',  ( -108.7640941326033328, -289.6947882137466763, -285.9992733807759464 ) ) ;
#26508=CARTESIAN_POINT ( 'NONE',  ( -107.5840519861814073, -285.7688144943634256, -249.4626722518927409 ) ) ;
#26509=CARTESIAN_POINT ( 'NONE',  ( -2.245378395762407386, -286.0116838537664421, -201.8790478997052560 ) ) ;
#26510=CARTESIAN_POINT ( 'NONE',  ( -29.97397971420965490, -124.9943380580637040, -364.2934218382724794 ) ) ;
#26511=CARTESIAN_POINT ( 'NONE',  ( 20.79876770051471979, -280.5858102905837654, -315.8157813100587532 ) ) ;
#26512=CARTESIAN_POINT ( 'NONE',  ( 33.84787573538152827, -289.1381919327232595, -249.2709037235404139 ) ) ;
#26513=CARTESIAN_POINT ( 'NONE',  ( -2.114097185898930586, -281.0567505037315641, -335.1036166233522522 ) ) ;
#26514=CARTESIAN_POINT ( 'NONE',  ( -109.7692447497787782, -279.7029641874109416, -282.9051393760942688 ) ) ;
#26515=CARTESIAN_POINT ( 'NONE',  ( 3.173436779058369073, -276.9837799162163492, -331.1600663529284816 ) ) ;
#26516=CARTESIAN_POINT ( 'NONE',  ( -81.68796297553329566, -290.2579340431400965, -207.8997884333085437 ) ) ;
#26518=CARTESIAN_POINT ( 'NONE',  ( -110.9503421328437156, -285.0772499776066979, -292.4505304951155154 ) ) ;
#26519=CARTESIAN_POINT ( 'NONE',  ( -110.8690832948050797, -285.3312678423222906, -247.5267119884094029 ) ) ;
#26520=CARTESIAN_POINT ( 'NONE',  ( 35.51973029490412870, -281.6595265698347248, -265.8653465021923807 ) ) ;
#26523=CARTESIAN_POINT ( 'NONE',  ( -111.7170394036605501, -292.5970046144173011, -255.8499364584392879 ) ) ;
#26524=CARTESIAN_POINT ( 'NONE',  ( -7.367873120264879283, -291.1218943247145035, -199.9560634122750855 ) ) ;
#26525=CARTESIAN_POINT ( 'NONE',  ( 35.58723100020613117, -274.6988866956650668, -277.0528630635745344 ) ) ;
#26526=CARTESIAN_POINT ( 'NONE',  ( -64.23831415584729143, -294.7426565363705322, -342.4019740322032135 ) ) ;
#26527=CARTESIAN_POINT ( 'NONE',  ( -36.17592627345034373, -290.5468699734470306, -196.6644088236953110 ) ) ;
#26528=CARTESIAN_POINT ( 'NONE',  ( -70.19373344906404100, -293.7310247842222566, -336.6839490670975579 ) ) ;
#26529=CARTESIAN_POINT ( 'NONE',  ( -84.93088073728347354, -290.9306001197653586, -326.3066328120752360 ) ) ;
#26531=CARTESIAN_POINT ( 'NONE',  ( -88.11823665433593078, -291.7630158053539162, -325.5584366206380196 ) ) ;
#26532=CARTESIAN_POINT ( 'NONE',  ( 21.68464018457738263, -290.9141717036186492, -223.8010994277454699 ) ) ;
#26533=CARTESIAN_POINT ( 'NONE',  ( -63.89893834446905174, -297.3984842723367024, -340.5564354515693708 ) ) ;
#26534=CARTESIAN_POINT ( 'NONE',  ( -46.76699100961059941, -286.8709478556596650, -197.6839273504741641 ) ) ;
#26535=CARTESIAN_POINT ( 'NONE',  ( 16.27219540724796332, -296.2938587505097985, -323.1189366517678536 ) ) ;
#26536=CARTESIAN_POINT ( 'NONE',  ( 25.54375624049132298, -276.9741158277753925, -228.8421322068949735 ) ) ;
#26537=CARTESIAN_POINT ( 'NONE',  ( 24.04023758294295376, -274.9599163340035943, -316.1897819657462492 ) ) ;
#26538=CARTESIAN_POINT ( 'NONE',  ( -46.10129540644673796, -297.1408961589830824, -194.0235236347846239 ) ) ;
#26539=CARTESIAN_POINT ( 'NONE',  ( 19.06636603510410666, -274.4640639476404544, -318.2787983033752539 ) ) ;
#26540=CARTESIAN_POINT ( 'NONE',  ( -86.41550047006222712, -277.4442672832196308, -214.3872283979690962 ) ) ;
#26541=CARTESIAN_POINT ( 'NONE',  ( -107.5809884703223531, -274.0397678758758389, -248.8896469012588852 ) ) ;
#26542=CARTESIAN_POINT ( 'NONE',  ( -106.5350642620218196, -297.6445838101986965, -295.5638594249705307 ) ) ;
#26544=CARTESIAN_POINT ( 'NONE',  ( 133.0872704186301405, -299.5541904835127980, -195.3611179825600175 ) ) ;
#26545=CARTESIAN_POINT ( 'NONE',  ( -108.9392745071751847, -297.5538113406017828, -255.2546091852232450 ) ) ;
#26546=DIRECTION ( 'NONE',  ( 0.000000000000000000, 0.000000000000000000, 1.000000000000000000 ) ) ;
#26547=CARTESIAN_POINT ( 'NONE',  ( 26.04724258167656714, -286.1196050401511570, -311.2034313418628244 ) ) ;
#26548=CARTESIAN_POINT ( 'NONE',  ( -33.81211282506870219, -298.0975490310236182, -197.3611180786018906 ) ) ;
#26549=CARTESIAN_POINT ( 'NONE',  ( 14.24688035217459614, -286.7531436488690701, -213.1264980538594784 ) ) ;
#26550=CARTESIAN_POINT ( 'NONE',  ( -99.85557839221172571, -289.6230742935561011, -315.3031793183994296 ) ) ;
#26551=CARTESIAN_POINT ( 'NONE',  ( -111.5244497003094040, -298.7012547784190701, -257.1200277484309709 ) ) ;
#26552=CARTESIAN_POINT ( 'NONE',  ( 35.85563456518634240, -291.7530438902615515, -285.9845753726145858 ) ) ;
#26553=CARTESIAN_POINT ( 'NONE',  ( 38.50679924301480384, -280.9044393674689104, -282.7381164179409438 ) ) ;
#26555=CARTESIAN_POINT ( 'NONE',  ( -103.2055037226382126, -277.0298764946494998, -234.3796325430344041 ) ) ;
#26557=CARTESIAN_POINT ( 'NONE',  ( -56.18224285526869011, -288.0950911280332321, -341.3517143386196722 ) ) ;
#26559=CARTESIAN_POINT ( 'NONE',  ( -109.6609731769846690, -288.2942020699566683, -290.4254254028564333 ) ) ;
#26560=CARTESIAN_POINT ( 'NONE',  ( 52.87650880464764214, -300.8000763623448961, -196.5360689618387653 ) ) ;
#26561=CARTESIAN_POINT ( 'NONE',  ( -5.682957858946411811, -284.0691747476666364, -339.9048476258201390 ) ) ;
#26562=CARTESIAN_POINT ( 'NONE',  ( -48.69670390260161241, -295.9284888967570737, -195.8138301115931199 ) ) ;
#26563=CARTESIAN_POINT ( 'NONE',  ( 5.592090758289988806, -282.4520845465209504, -329.4008469802894297 ) ) ;
#26564=CARTESIAN_POINT ( 'NONE',  ( -68.54883825244230877, -275.0591516243557066, -203.7028078640957744 ) ) ;
#26566=CARTESIAN_POINT ( 'NONE',  ( 2.731262588749159725, -282.5894332169731342, -206.9029527851270132 ) ) ;
#26567=CARTESIAN_POINT ( 'NONE',  ( -99.53548307293127095, -272.0058865167704880, -231.5518480033855440 ) ) ;
#26570=CARTESIAN_POINT ( 'NONE',  ( -97.92420053106265243, -287.1286239239596512, -226.7318789255200215 ) ) ;
#26572=CARTESIAN_POINT ( 'NONE',  ( -72.08107566293803359, -274.9809262143061233, -342.4248175857292154 ) ) ;
#26573=CARTESIAN_POINT ( 'NONE',  ( -93.22359948505962279, -277.0270378273148140, -323.1761956177509774 ) ) ;
#26574=CARTESIAN_POINT ( 'NONE',  ( -69.04326074436966110, -287.8620039541802953, -339.6679004253663265 ) ) ;
#26575=CARTESIAN_POINT ( 'NONE',  ( -70.50980722328270645, -285.0177218327364699, -336.1824039134395434 ) ) ;
#26577=CARTESIAN_POINT ( 'NONE',  ( -5.825046441744500036, -278.3921525149904141, -337.3427927951235574 ) ) ;
#26578=CARTESIAN_POINT ( 'NONE',  ( -113.6188819958375831, -285.9102025247194092, -275.6948728675853886 ) ) ;
#26579=CARTESIAN_POINT ( 'NONE',  ( -51.10733440467242161, -282.0268015300047182, -342.5076214538783574 ) ) ;
#26580=CARTESIAN_POINT ( 'NONE',  ( 29.55406908845921521, -283.1027979530119296, -236.3350273926781995 ) ) ;
#26581=CARTESIAN_POINT ( 'NONE',  ( -26.99862114891847753, -274.3467363944650970, -194.0055208881272790 ) ) ;
#26582=CARTESIAN_POINT ( 'NONE',  ( -109.7374885423401309, -278.0524649331115370, -296.7439976247471805 ) ) ;
#26583=CARTESIAN_POINT ( 'NONE',  ( -108.9821371495358875, -298.2101449321713744, -290.5839264639818680 ) ) ;
#26586=CARTESIAN_POINT ( 'NONE',  ( -113.1025904759236056, -294.7015227549535439, -269.5910715669770639 ) ) ;
#26587=CARTESIAN_POINT ( 'NONE',  ( 16.57233386806656128, -275.7667254891260882, -319.6876392050527329 ) ) ;
#26588=CARTESIAN_POINT ( 'NONE',  ( -95.73501774525767871, -274.4292146643537080, -220.7603842714128746 ) ) ;
#26589=CARTESIAN_POINT ( 'NONE',  ( 13.82411070878751325, -288.5412276956427604, -216.8111478844424767 ) ) ;
#26590=CARTESIAN_POINT ( 'NONE',  ( -2.268766472257749189, -296.1165910632869327, -338.1298207832799676 ) ) ;
#26591=CARTESIAN_POINT ( 'NONE',  ( 6.399918719456080041, -295.6778618717204381, -333.3120023830723540 ) ) ;
#26592=CARTESIAN_POINT ( 'NONE',  ( -106.4046333997188043, -292.9309371335982064, -241.4105453432695469 ) ) ;
#26593=CARTESIAN_POINT ( 'NONE',  ( -102.3932453609285744, -277.0462243160820321, -233.3702422569386954 ) ) ;
#26594=CARTESIAN_POINT ( 'NONE',  ( -54.85483508047848744, -281.7455735179509588, -197.9573212376795084 ) ) ;
#26595=CARTESIAN_POINT ( 'NONE',  ( -81.01906985839417530, -293.7304093400820761, -330.6404806920920691 ) ) ;
#26596=CARTESIAN_POINT ( 'NONE',  ( -94.38882485583700088, -285.7271955080646535, -320.2202299134325472 ) ) ;
#26597=CARTESIAN_POINT ( 'NONE',  ( -93.48299884858347752, -284.1391430164480880, -223.2189855270897851 ) ) ;
#26598=CARTESIAN_POINT ( 'NONE',  ( -46.16520984643562997, -156.0173353556437803, -364.2845566487454789 ) ) ;
#26600=CARTESIAN_POINT ( 'NONE',  ( -52.08905897353218961, -285.5248435149476336, -198.8446660727839230 ) ) ;
#26602=CARTESIAN_POINT ( 'NONE',  ( 37.25094498424395084, -282.8561927816836032, -288.2337364978654932 ) ) ;
#26603=CARTESIAN_POINT ( 'NONE',  ( -51.56973345032491096, -274.1985478715116642, -198.6877339617595339 ) ) ;
#26604=CARTESIAN_POINT ( 'NONE',  ( -64.39254046066720605, -284.5017778985966288, -198.6793139480549542 ) ) ;
#26605=CARTESIAN_POINT ( 'NONE',  ( -50.90985073277121842, -280.8240876805172661, -194.8050096821539512 ) ) ;
#26607=CARTESIAN_POINT ( 'NONE',  ( -81.85028284571910717, -280.9779593741140502, -208.3797190346592174 ) ) ;
#26608=CARTESIAN_POINT ( 'NONE',  ( -4.994423991111502481, -281.1183700868226651, -200.5974704747835631 ) ) ;
#26609=CARTESIAN_POINT ( 'NONE',  ( 30.91033621190086578, -278.8380690714489560, -254.8156830097664738 ) ) ;
#26610=CARTESIAN_POINT ( 'NONE',  ( 203.1353409855606174, 293.1658297356431717, -83.22860506881615095 ) ) ;
#26612=CARTESIAN_POINT ( 'NONE',  ( 10.64158200923520603, -276.7166477349687739, -212.8682576112067864 ) ) ;
#26613=CARTESIAN_POINT ( 'NONE',  ( 199.2237029682673040, 289.5565456333249585, -97.44563473156274824 ) ) ;
#26614=CARTESIAN_POINT ( 'NONE',  ( -107.9935472655180035, -276.8871626603749405, -246.1159714119290243 ) ) ;
#26615=CARTESIAN_POINT ( 'NONE',  ( -35.01420788653632599, -293.8411093123329465, -194.3971249997707389 ) ) ;
#26616=CARTESIAN_POINT ( 'NONE',  ( -100.2584255176955423, -295.3888303900021697, -307.6814793703455280 ) ) ;
#26617=CARTESIAN_POINT ( 'NONE',  ( -108.3079553782693267, -290.4381402463579889, -240.6404598667304811 ) ) ;
#26619=CARTESIAN_POINT ( 'NONE',  ( -90.31674821449534818, -294.3584517662027338, -325.4998569303264162 ) ) ;
#26620=CARTESIAN_POINT ( 'NONE',  ( 34.78828026051343159, -286.1564502513272714, -286.0314063445531474 ) ) ;
#26621=CARTESIAN_POINT ( 'NONE',  ( 21.51680376796998573, -296.0388320105424782, -315.6206612025129061 ) ) ;
#26622=CARTESIAN_POINT ( 'NONE',  ( 36.04617335688610780, -286.1742074106616087, -265.5711379855692940 ) ) ;
#26623=CARTESIAN_POINT ( 'NONE',  ( -110.1028095986347921, -286.0029120330531214, -260.0139238334185166 ) ) ;
#26624=CARTESIAN_POINT ( 'NONE',  ( -36.39335253043677199, -293.0050168633503063, -193.5892769763656815 ) ) ;
#26625=CARTESIAN_POINT ( 'NONE',  ( 1.139045458816819067, -283.0159751336047975, -332.5267231827461387 ) ) ;
#26627=CARTESIAN_POINT ( 'NONE',  ( -74.42764890964282642, -294.3286134549203439, -337.4476952199739230 ) ) ;
#26628=CARTESIAN_POINT ( 'NONE',  ( -98.22659652858438051, -291.9819867019043045, -223.4656495923142643 ) ) ;
#26629=CARTESIAN_POINT ( 'NONE',  ( -99.81662905474614433, -290.4485692968793842, -315.2881433868143972 ) ) ;
#26630=CARTESIAN_POINT ( 'NONE',  ( 9.028855969126675873, -286.8762175665992800, -213.9805226352355021 ) ) ;
#26633=CARTESIAN_POINT ( 'NONE',  ( -112.1733633310270619, -298.5642851474183317, -258.4243337670610572 ) ) ;
#26634=CARTESIAN_POINT ( 'NONE',  ( -40.40363980321603776, -296.6993820149667727, -193.8637701130283233 ) ) ;
#26636=CARTESIAN_POINT ( 'NONE',  ( 11.47153953092307788, -279.8079787482593588, -215.7655496504346502 ) ) ;
#26638=CARTESIAN_POINT ( 'NONE',  ( 39.56160809400698497, -275.1059432973352727, -274.0472738088151345 ) ) ;
#26639=CARTESIAN_POINT ( 'NONE',  ( -47.34791026978283668, -296.4027107693032690, -197.2985773678334454 ) ) ;
#26640=CARTESIAN_POINT ( 'NONE',  ( -64.76781208370880449, -279.2744307884012187, -339.3988418925890187 ) ) ;
#26641=CARTESIAN_POINT ( 'NONE',  ( -3.521145360883818132, -272.6430019281157797, -204.2632959257987864 ) ) ;
#26642=CARTESIAN_POINT ( 'NONE',  ( -94.24067830949607583, -297.1042624233357401, -316.7450419354605060 ) ) ;
#26643=CARTESIAN_POINT ( 'NONE',  ( -37.16260514514985402, -299.1341274580777849, -197.0491090442832274 ) ) ;
#26645=CARTESIAN_POINT ( 'NONE',  ( -2.316862567297136799, -296.1965845442257432, -338.0346074098131339 ) ) ;
#26646=CARTESIAN_POINT ( 'NONE',  ( -26.51331991724878634, -296.1872443344852286, -195.1981240880892585 ) ) ;
#26647=CARTESIAN_POINT ( 'NONE',  ( -64.11665814124751250, -292.3448467768403702, -202.3255520286885769 ) ) ;
#26648=CARTESIAN_POINT ( 'NONE',  ( -92.99027580637627466, -289.8075467350213330, -222.2091611867411132 ) ) ;
#26650=CARTESIAN_POINT ( 'NONE',  ( 26.09027815450861354, -275.4691217511748960, -226.7957087249940287 ) ) ;
#26651=CARTESIAN_POINT ( 'NONE',  ( -88.14350127068128415, -297.6506479540262262, -217.8380217683297531 ) ) ;
#26652=CARTESIAN_POINT ( 'NONE',  ( 30.52883827193004507, -283.1014426512995783, -237.4997932801988156 ) ) ;
#26654=CARTESIAN_POINT ( 'NONE',  ( 33.87157781651384880, -279.8785624894327384, -242.2527628918645064 ) ) ;
#26655=CARTESIAN_POINT ( 'NONE',  ( -51.30226326775083123, -276.5747454194122952, -345.9813233718141987 ) ) ;
#26656=CARTESIAN_POINT ( 'NONE',  ( -33.49794300959267446, -282.1997323130977406, -343.4341540528075143 ) ) ;
#26657=CARTESIAN_POINT ( 'NONE',  ( 35.41078938508652385, -279.7942832994010587, -289.2583055848575668 ) ) ;
#26659=CARTESIAN_POINT ( 'NONE',  ( -29.91247694883873365, -272.7227504864325738, -197.1478571631043621 ) ) ;
#26660=CARTESIAN_POINT ( 'NONE',  ( -110.5025717868261950, -280.7649202286031596, -253.7968955414481229 ) ) ;
#26663=CARTESIAN_POINT ( 'NONE',  ( -77.64574571157193361, -295.7588089152417297, -205.9440556284513661 ) ) ;
#26664=CARTESIAN_POINT ( 'NONE',  ( -110.4309002539738032, -290.8589900752696167, -245.9668213614052661 ) ) ;
#26665=CARTESIAN_POINT ( 'NONE',  ( 31.35481885158082704, -277.9511857978322382, -300.8704067920850775 ) ) ;
#26666=CARTESIAN_POINT ( 'NONE',  ( 16.91066350521142070, -272.8242979144282572, -218.5009557823775310 ) ) ;
#26668=CARTESIAN_POINT ( 'NONE',  ( -102.8053316724463855, -286.9733583429897976, -232.5233784389450307 ) ) ;
#26671=CARTESIAN_POINT ( 'NONE',  ( 28.08357908928204694, -286.0414683489416916, -307.1334348813559245 ) ) ;
#26673=CARTESIAN_POINT ( 'NONE',  ( -15.48916135804726935, -293.5579849021808059, -340.4830915405719338 ) ) ;
#26674=CARTESIAN_POINT ( 'NONE',  ( 14.01083334673153935, -284.9212536848378363, -216.6825002618953135 ) ) ;
#26675=CARTESIAN_POINT ( 'NONE',  ( 20.69763459394507876, -20.92298310053570987, -343.0354172471594438 ) ) ;
#26676=CARTESIAN_POINT ( 'NONE',  ( -28.68987852629980395, -292.9424050472306931, -344.9128340944349702 ) ) ;
#26677=CARTESIAN_POINT ( 'NONE',  ( -5.049601808426840144, -284.9494797728412436, -201.2240935930309718 ) ) ;
#26678=CARTESIAN_POINT ( 'NONE',  ( -109.6753821937728333, -280.3441219744390764, -255.6593066754535073 ) ) ;
#26679=CARTESIAN_POINT ( 'NONE',  ( 37.63169741978722271, -288.5588532396723167, -254.5814832043031402 ) ) ;
#26680=CARTESIAN_POINT ( 'NONE',  ( 35.63291226925915822, -279.5223145476238074, -249.1323558094555608 ) ) ;
#26681=CARTESIAN_POINT ( 'NONE',  ( -58.68913036541010086, -289.3359118507994481, -340.2228556556863737 ) ) ;
#26682=CARTESIAN_POINT ( 'NONE',  ( -79.40642690274627569, -280.8968608245478435, -209.9795506195519010 ) ) ;
#26683=CARTESIAN_POINT ( 'NONE',  ( -57.16676531630589864, -280.5925665085519540, -199.9369139275347891 ) ) ;
#26685=CARTESIAN_POINT ( 'NONE',  ( -80.02770050428505044, -287.4579966027558271, -208.1989085970629105 ) ) ;
#26687=CARTESIAN_POINT ( 'NONE',  ( -85.80823110288866928, -273.4019493347999514, -210.5280554229012182 ) ) ;
#26688=CARTESIAN_POINT ( 'NONE',  ( -106.2305628964040380, -292.9106721050465012, -241.4833040373116830 ) ) ;
#26690=CARTESIAN_POINT ( 'NONE',  ( -72.02372285203398405, -297.9805209788416391, -342.4524372437778652 ) ) ;
#26692=CARTESIAN_POINT ( 'NONE',  ( 10.63557830801703474, -272.7126596835998953, -212.4297516463423960 ) ) ;
#26694=CARTESIAN_POINT ( 'NONE',  ( -109.5937020379772093, -294.6439827360587174, -294.5703855230362365 ) ) ;
#26695=CARTESIAN_POINT ( 'NONE',  ( -105.8613594928522588, -296.3993908458012925, -244.8568972348122941 ) ) ;
#26696=CARTESIAN_POINT ( 'NONE',  ( -31.80007785805864629, -290.5012212748150091, -343.8969021430283988 ) ) ;
#26697=CARTESIAN_POINT ( 'NONE',  ( 21.83340476600337965, -283.9281828454697916, -314.8374508501866558 ) ) ;
#26698=CARTESIAN_POINT ( 'NONE',  ( -48.76286128286598398, -290.6200099286714362, -345.9670361056142838 ) ) ;
#26699=CARTESIAN_POINT ( 'NONE',  ( -112.4441006938225911, -292.0518508526362780, -255.7007530701744145 ) ) ;
#26700=CARTESIAN_POINT ( 'NONE',  ( -22.07700354926762998, -288.2477330005200429, -196.8776510896352363 ) ) ;
#26701=CARTESIAN_POINT ( 'NONE',  ( -79.91254976740866312, -279.6605278899509699, -206.1354645271921413 ) ) ;
#26702=CARTESIAN_POINT ( 'NONE',  ( -111.9634914974103737, -294.7843254702183913, -258.4090831289626067 ) ) ;
#26703=CARTESIAN_POINT ( 'NONE',  ( -70.47204212879293550, -283.3101654618914722, -339.8837119342994697 ) ) ;
#26704=CARTESIAN_POINT ( 'NONE',  ( 35.93017762072240373, -277.5712424504486648, -282.5927812587456174 ) ) ;
#26706=CARTESIAN_POINT ( 'NONE',  ( -37.37352853689063892, -300.5519495502701943, -195.3611179825600175 ) ) ;
#26707=CARTESIAN_POINT ( 'NONE',  ( 35.90279160379202494, -274.0493711301563167, -290.6387294181315042 ) ) ;
#26708=CARTESIAN_POINT ( 'NONE',  ( 128.9467878515196162, -299.5541904835127980, -200.7046326357662167 ) ) ;
#26709=CARTESIAN_POINT ( 'NONE',  ( 33.70852362246065326, -281.2849055538088692, -287.4394281841307475 ) ) ;
#26710=CARTESIAN_POINT ( 'NONE',  ( -113.9808707652687332, -279.7773802568665928, -268.7579503831991019 ) ) ;
#26711=CARTESIAN_POINT ( 'NONE',  ( -60.42770478585716631, -284.8187905249547498, -197.0946735001964782 ) ) ;
#26712=CARTESIAN_POINT ( 'NONE',  ( 31.76667377241848556, -294.9632711882800891, -243.8657095369515844 ) ) ;
#26713=CARTESIAN_POINT ( 'NONE',  ( -103.5446941996294612, -274.6486547209605078, -232.5245009089235282 ) ) ;
#26714=CARTESIAN_POINT ( 'NONE',  ( -67.35769383500377216, -274.9818023116616246, -199.9882652951150135 ) ) ;
#26715=DIRECTION ( 'NONE',  ( -1.000000000000000000, -0.000000000000000000, -0.000000000000000000 ) ) ;
#26716=CARTESIAN_POINT ( 'NONE',  ( 29.15339240532204101, -275.7914696594816064, -300.4842432098263885 ) ) ;
#26717=CARTESIAN_POINT ( 'NONE',  ( -103.0656304090098558, -298.0758436247911050, -306.1437033027143002 ) ) ;
#26718=CARTESIAN_POINT ( 'NONE',  ( -98.04749957200297672, -283.1492142525569307, -226.5804470698925570 ) ) ;
#26719=CARTESIAN_POINT ( 'NONE',  ( 39.20557941290697812, -293.1109296196158880, -261.7325060403586008 ) ) ;
#26720=CARTESIAN_POINT ( 'NONE',  ( 28.09020284683080249, -273.0911317999635344, -234.3296155778404568 ) ) ;
#26721=CARTESIAN_POINT ( 'NONE',  ( 0.3415919811142267837, -290.1594153328171615, -336.6507297303911059 ) ) ;
#26722=CARTESIAN_POINT ( 'NONE',  ( 30.14567044497053061, -292.0881689145955420, -241.6011181777199681 ) ) ;
#26724=CARTESIAN_POINT ( 'NONE',  ( 8.511947109087856234, -291.2407382222393153, -209.1718393089742563 ) ) ;
#26726=CARTESIAN_POINT ( 'NONE',  ( -101.1400853280757275, -290.7056938149839880, -234.7346959321048416 ) ) ;
#26727=ORIENTED_EDGE ( 'NONE', *, *, #18614, .T. ) ;
#26728=CARTESIAN_POINT ( 'NONE',  ( 19.40482051515830619, -289.3359029226850794, -321.9687132998352581 ) ) ;
#26729=CARTESIAN_POINT ( 'NONE',  ( -109.9876022629710519, -278.9893312455164960, -262.4829533495619671 ) ) ;
#26730=CARTESIAN_POINT ( 'NONE',  ( -47.60387215835924479, -294.1000392679046058, -346.3623043837709474 ) ) ;
#26731=CARTESIAN_POINT ( 'NONE',  ( -57.73689604186656510, -286.4470393917743536, -196.1617298398948037 ) ) ;
#26732=CARTESIAN_POINT ( 'NONE',  ( -114.3336063875097039, -284.8542623932090123, -272.8527847642692450 ) ) ;
#26733=CARTESIAN_POINT ( 'NONE',  ( -61.53772696028209310, -283.7084779206152803, -339.3102300259312756 ) ) ;
#26734=CARTESIAN_POINT ( 'NONE',  ( 202.2819390781037328, 293.6457075726772246, -83.22913366109028743 ) ) ;
#26735=CARTESIAN_POINT ( 'NONE',  ( -114.3334814850269652, -272.1971439235380785, -284.0165574570778517 ) ) ;
#26736=CARTESIAN_POINT ( 'NONE',  ( 178.3113800505042263, 252.0692767011776141, -164.4075532967166282 ) ) ;
#26738=CARTESIAN_POINT ( 'NONE',  ( 32.66794128697139143, -275.0304942085265907, -291.6472148795279509 ) ) ;
#26739=CARTESIAN_POINT ( 'NONE',  ( 35.00997217543812212, -274.6316298465533237, -282.4768840196937276 ) ) ;
#26740=CARTESIAN_POINT ( 'NONE',  ( -113.8826363757102342, -295.9620406538865609, -278.1721346557389438 ) ) ;
#26741=CARTESIAN_POINT ( 'NONE',  ( 168.6450565192255908, 229.6397774369325191, -190.3058657457524987 ) ) ;
#26742=CARTESIAN_POINT ( 'NONE',  ( 5.580683173876516356, -275.1687501424511311, -333.6933158240120747 ) ) ;
#26743=CARTESIAN_POINT ( 'NONE',  ( -109.5281245247177395, -274.5249336607064379, -254.0181026674689235 ) ) ;
#26745=CARTESIAN_POINT ( 'NONE',  ( -68.09424279708272820, -298.5995022204775182, -199.9688556016709242 ) ) ;
#26746=CARTESIAN_POINT ( 'NONE',  ( 12.20213218960536317, -288.8329435094427140, -324.1271433072680566 ) ) ;
#26747=CARTESIAN_POINT ( 'NONE',  ( -37.67798924117062143, -295.8590548613066176, -347.2119575608210198 ) ) ;
#26748=CARTESIAN_POINT ( 'NONE',  ( -114.1719552471954842, -296.9821601478535058, -275.3416426531995285 ) ) ;
#26749=CARTESIAN_POINT ( 'NONE',  ( -20.07422210092791559, -292.4468366246763935, -199.3804751816619785 ) ) ;
#26751=CARTESIAN_POINT ( 'NONE',  ( 36.53225936691014653, -277.2692256905613704, -254.4270362188295564 ) ) ;
#26754=CARTESIAN_POINT ( 'NONE',  ( 38.73484462456460165, -280.9117392967417004, -258.5312220010501392 ) ) ;
#26755=CARTESIAN_POINT ( 'NONE',  ( -8.635436142503104762, -277.6082965895639063, -337.7494695137468739 ) ) ;
#26756=CARTESIAN_POINT ( 'NONE',  ( -28.69380377777484981, -278.7042004190103626, -345.9069553965588852 ) ) ;
#26757=CARTESIAN_POINT ( 'NONE',  ( -53.79716647774889537, -275.2822944587104530, -343.9511463772141724 ) ) ;
#26758=CARTESIAN_POINT ( 'NONE',  ( -75.27061711250985354, -298.1838275818548141, -207.8101070488927178 ) ) ;
#26759=CARTESIAN_POINT ( 'NONE',  ( -109.9472088980176352, -294.9699439457618269, -282.3534077577143080 ) ) ;
#26761=CARTESIAN_POINT ( 'NONE',  ( -69.94201088550713052, -280.1265866060051621, -200.6563771082540200 ) ) ;
#26762=CARTESIAN_POINT ( 'NONE',  ( 13.73284503741700924, -276.4787771678597323, -322.5888861671180621 ) ) ;
#26763=CARTESIAN_POINT ( 'NONE',  ( 18.27474897256593067, -286.9591091875677193, -322.8978561957890747 ) ) ;
#26764=CARTESIAN_POINT ( 'NONE',  ( -43.17355122162680203, -299.9789741424969520, -195.3690785949184487 ) ) ;
#26765=CARTESIAN_POINT ( 'NONE',  ( 82.61703178011177329, -302.0572532870764917, -195.4731947519462381 ) ) ;
#26766=CARTESIAN_POINT ( 'NONE',  ( 21.29679143005557762, -287.3620939802576686, -314.1328459475130899 ) ) ;
#26767=CARTESIAN_POINT ( 'NONE',  ( 7.777565281487036408, -278.9173574572075722, -211.6257724223393950 ) ) ;
#26768=CARTESIAN_POINT ( 'NONE',  ( -98.47304628710297436, -277.6924307189788692, -229.3031982849115877 ) ) ;
#26769=CARTESIAN_POINT ( 'NONE',  ( -54.03593491015463712, -281.3478465225171021, -342.9581291951858475 ) ) ;
#26770=CARTESIAN_POINT ( 'NONE',  ( 19.78164113593015472, -288.8793855325270101, -221.7419617896272257 ) ) ;
#26771=CARTESIAN_POINT ( 'NONE',  ( -109.5253815661579750, -279.9316113518907514, -257.0702700157197569 ) ) ;
#26773=CARTESIAN_POINT ( 'NONE',  ( 9.840308027229815124, -294.7015614803166841, -211.9945877116911674 ) ) ;
#26774=CARTESIAN_POINT ( 'NONE',  ( -111.5004251917811757, -276.5820645079326141, -286.9278773107641882 ) ) ;
#26775=CARTESIAN_POINT ( 'NONE',  ( -35.10621908121218837, -277.6747570548651538, -343.4288625280283327 ) ) ;
#26776=CARTESIAN_POINT ( 'NONE',  ( -0.01927517540570689372, -284.5569116127358598, -335.6221778246190297 ) ) ;
#26778=CARTESIAN_POINT ( 'NONE',  ( -51.39309154084573095, -291.1506368762147190, -344.6031047197599264 ) ) ;
#26779=CARTESIAN_POINT ( 'NONE',  ( -93.43172067399453340, -295.2448062213551339, -220.5533411413741192 ) ) ;
#26780=CARTESIAN_POINT ( 'NONE',  ( -68.42604364488623503, -284.8512438904770647, -200.0764205640718671 ) ) ;
#26782=CARTESIAN_POINT ( 'NONE',  ( -74.50841538816288789, -272.2318228359258114, -206.8996594922552390 ) ) ;
#26783=CARTESIAN_POINT ( 'NONE',  ( -32.04591552392162157, -290.2592168845200717, -196.3022163802394289 ) ) ;
#26786=CARTESIAN_POINT ( 'NONE',  ( -25.11330357806730618, -290.6852544266612313, -195.0406422206420416 ) ) ;
#26787=CARTESIAN_POINT ( 'NONE',  ( -100.3023504785266908, -286.6781908489620605, -231.7618021565259596 ) ) ;
#26788=CARTESIAN_POINT ( 'NONE',  ( 21.32233432843219134, -285.1345184668953721, -222.0651028445196857 ) ) ;
#26789=CARTESIAN_POINT ( 'NONE',  ( -65.33403583430848016, -287.1043540183163714, -202.2495104004988491 ) ) ;
#26791=CARTESIAN_POINT ( 'NONE',  ( -22.43690667272922923, -287.0505977705300893, -198.6819724489680823 ) ) ;
#26792=CARTESIAN_POINT ( 'NONE',  ( -14.39190050869001070, -294.3280006531069830, -198.5309070168546839 ) ) ;
#26793=CARTESIAN_POINT ( 'NONE',  ( 35.10569085269639089, -273.9069397194713247, -291.8704007981729092 ) ) ;
#26794=CARTESIAN_POINT ( 'NONE',  ( 38.16245962426862803, -276.0730230554119657, -285.3566557088650484 ) ) ;
#26795=CARTESIAN_POINT ( 'NONE',  ( -9.027696117552387989, -290.4994204145099843, -200.3066293631628128 ) ) ;
#26796=CARTESIAN_POINT ( 'NONE',  ( -112.4844053670614841, -278.3419207576978920, -287.1710510391713456 ) ) ;
#26797=CARTESIAN_POINT ( 'NONE',  ( -110.6660317147119201, -298.7132563259610833, -256.3147549761018809 ) ) ;
#26800=CARTESIAN_POINT ( 'NONE',  ( -107.4613583187515502, -282.9471993809232231, -292.3719565269367990 ) ) ;
#26801=CARTESIAN_POINT ( 'NONE',  ( 11.70403046443786543, -278.7329559851858107, -213.6203305672067643 ) ) ;
#26803=CARTESIAN_POINT ( 'NONE',  ( 23.09566817772254765, -273.4044882982954618, -223.7562380433323597 ) ) ;
#26804=CARTESIAN_POINT ( 'NONE',  ( -70.50644846288548706, -276.8500975787258085, -335.5070475284564964 ) ) ;
#26805=CARTESIAN_POINT ( 'NONE',  ( -28.79654450267103272, -296.4621202232191877, -343.6088471089033192 ) ) ;
#26806=CARTESIAN_POINT ( 'NONE',  ( 19.90713851165421744, -279.7777003198740999, -219.3113472844424336 ) ) ;
#26807=CARTESIAN_POINT ( 'NONE',  ( -84.62089232753784529, -296.6632429145123524, -326.3569905383864693 ) ) ;
#26808=CARTESIAN_POINT ( 'NONE',  ( -99.59738945185569037, -297.2734305052078980, -314.9197229273113408 ) ) ;
#26809=CARTESIAN_POINT ( 'NONE',  ( -94.62665685498387802, -272.8576989399874719, -225.0784367492727256 ) ) ;
#26810=CARTESIAN_POINT ( 'NONE',  ( -110.6712509847548915, -292.7544217102014841, -254.6201642601380684 ) ) ;
#26811=CARTESIAN_POINT ( 'NONE',  ( -109.0292583420370107, -285.0767217503002371, -242.1110506428756821 ) ) ;
#26812=CARTESIAN_POINT ( 'NONE',  ( -4.551223575848055702, -274.7643480253225334, -338.6768466695388611 ) ) ;
#26813=CARTESIAN_POINT ( 'NONE',  ( 37.50391401686425041, -287.6123362159589760, -288.5036594769578642 ) ) ;
#26814=CARTESIAN_POINT ( 'NONE',  ( -38.40199223413036833, -282.0186904250356861, -195.7111638853811257 ) ) ;
#26816=CARTESIAN_POINT ( 'NONE',  ( 19.70600566168781143, -285.9635036919077606, -224.4177466393263671 ) ) ;
#26817=CARTESIAN_POINT ( 'NONE',  ( -37.75769415766401238, -290.0467844270335718, -195.3622673089417106 ) ) ;
#26818=CARTESIAN_POINT ( 'NONE',  ( 143.8719904363247224, 176.7915900130879550, -240.1109971732525139 ) ) ;
#26819=CARTESIAN_POINT ( 'NONE',  ( 2.485805911679377367, -286.1097186457844828, -209.1095204178920142 ) ) ;
#26821=CARTESIAN_POINT ( 'NONE',  ( -112.6916892114120969, -289.7957896498892865, -255.6230206211112659 ) ) ;
#26822=CARTESIAN_POINT ( 'NONE',  ( -31.15920254897837438, -281.7290107928711791, -194.3601949015528874 ) ) ;
#26823=CARTESIAN_POINT ( 'NONE',  ( -113.2301690418536708, -279.9945947957406815, -260.2497534472397547 ) ) ;
#26824=CARTESIAN_POINT ( 'NONE',  ( 33.76087186793013473, -281.1673367844774134, -253.8255726304529674 ) ) ;
#26825=CARTESIAN_POINT ( 'NONE',  ( -1.992923467461159781, -276.5204772878800554, -204.2138229537782479 ) ) ;
#26826=CARTESIAN_POINT ( 'NONE',  ( -22.09754671479725729, -294.8620415794547966, -345.8370465075689708 ) ) ;
#26827=CARTESIAN_POINT ( 'NONE',  ( -93.78404694279149112, -289.2530164745510319, -221.5133105489995557 ) ) ;
#26828=CARTESIAN_POINT ( 'NONE',  ( -103.5567290587240592, -271.7730163139419233, -238.6956723466515768 ) ) ;
#26830=CARTESIAN_POINT ( 'NONE',  ( -92.72027240347070176, -285.7738895905237086, -320.1249180760857485 ) ) ;
#26831=CARTESIAN_POINT ( 'NONE',  ( 37.45675393577254653, -294.4185431453886395, -253.3705475995725465 ) ) ;
#26832=CARTESIAN_POINT ( 'NONE',  ( 19.43645414211531275, -282.8543406865946395, -316.4257628595906340 ) ) ;
#26833=CARTESIAN_POINT ( 'NONE',  ( 15.87258305593260488, -273.8429382517226145, -215.0342684632966836 ) ) ;
#26834=CARTESIAN_POINT ( 'NONE',  ( -111.8977884956055959, -291.4401261739023425, -251.4745095140122260 ) ) ;
#26835=CARTESIAN_POINT ( 'NONE',  ( -18.46647227692133697, -284.4322324114499452, -196.9309369347271002 ) ) ;
#26836=CARTESIAN_POINT ( 'NONE',  ( 19.39720699260034564, -293.1774582755224401, -218.3376549078637368 ) ) ;
#26837=CARTESIAN_POINT ( 'NONE',  ( 28.82732507518608855, -287.4685382405709788, -239.4783138623467664 ) ) ;
#26840=CARTESIAN_POINT ( 'NONE',  ( -47.25908889419609693, -155.3473324462872256, -361.3472553374705853 ) ) ;
#26841=CARTESIAN_POINT ( 'NONE',  ( -96.62141794101545145, -285.4217361794195540, -318.4297758286915609 ) ) ;
#26842=CARTESIAN_POINT ( 'NONE',  ( -95.99890600148557951, -281.4094976428775681, -317.0979686699210447 ) ) ;
#26844=CARTESIAN_POINT ( 'NONE',  ( 25.40796231749686385, -279.9517827164313530, -232.3588101084200730 ) ) ;
#26845=CARTESIAN_POINT ( 'NONE',  ( -35.71621215618927181, -276.6990367714955710, -347.3359302886096316 ) ) ;
#26846=CARTESIAN_POINT ( 'NONE',  ( -11.12412658756482209, -282.3946609980220046, -200.2159046499775741 ) ) ;
#26847=CARTESIAN_POINT ( 'NONE',  ( -53.93747043463056201, -170.5330345533709817, -362.6169925651183803 ) ) ;
#26848=CARTESIAN_POINT ( 'NONE',  ( 20.63100012324902721, -279.4496711621522422, -220.5639895147556047 ) ) ;
#26849=CARTESIAN_POINT ( 'NONE',  ( -42.76911677567638748, -284.0034641821418973, -195.9009786142026712 ) ) ;
#26850=CARTESIAN_POINT ( 'NONE',  ( -111.2934068659050553, -298.5336694902977115, -252.8934596384129350 ) ) ;
#26851=CARTESIAN_POINT ( 'NONE',  ( 16.20850676895009101, -294.7582654708452310, -320.0638722622853152 ) ) ;
#26853=CARTESIAN_POINT ( 'NONE',  ( -70.42783299816018427, -290.2912985678847804, -204.7367986250583840 ) ) ;
#26854=CARTESIAN_POINT ( 'NONE',  ( 19.80701368685719288, -276.9030616083088603, -321.8331081465513535 ) ) ;
#26855=CARTESIAN_POINT ( 'NONE',  ( -39.17045607675562024, -298.1952824628344842, -197.3716191773571040 ) ) ;
#26857=CARTESIAN_POINT ( 'NONE',  ( -95.78317314525202164, -272.1448369148741904, -220.6811935807979239 ) ) ;
#26858=DIRECTION ( 'NONE',  ( 0.000000000000000000, -1.000000000000000000, 0.000000000000000000 ) ) ;
#26861=CARTESIAN_POINT ( 'NONE',  ( 21.26527303377238809, -283.2478230585751930, -314.4210398522913579 ) ) ;
#26862=CARTESIAN_POINT ( 'NONE',  ( 38.39983156410941945, -283.2350025256452000, -264.2623977158010575 ) ) ;
#26863=CARTESIAN_POINT ( 'NONE',  ( -107.5772015095370904, -283.8866144012503128, -249.4396665204372709 ) ) ;
#26864=CARTESIAN_POINT ( 'NONE',  ( 35.89741892663457179, -274.0758245481443964, -279.8491786707871256 ) ) ;
#26865=CARTESIAN_POINT ( 'NONE',  ( 24.70206849985540387, -282.8557346562886323, -229.5077386161238167 ) ) ;
#26866=CARTESIAN_POINT ( 'NONE',  ( 34.25557951501436094, -274.2607410098478340, -287.8652135231621969 ) ) ;
#26867=EDGE_CURVE ( 'NONE', #44141, #34864, #11218, .T. ) ;
#26869=CARTESIAN_POINT ( 'NONE',  ( 29.36161962560460381, -276.2220507363093702, -239.8263110182279831 ) ) ;
#26871=CARTESIAN_POINT ( 'NONE',  ( -104.8288747155036305, -278.8785657172734886, -307.0985659920087301 ) ) ;
#26872=ORIENTED_EDGE ( 'NONE', *, *, #27217, .T. ) ;
#26875=CARTESIAN_POINT ( 'NONE',  ( -112.6731653155462993, -286.3097194944880926, -278.4528317648333200 ) ) ;
#26876=CARTESIAN_POINT ( 'NONE',  ( -88.62230904007013521, -294.9910732068373704, -322.6137471060431494 ) ) ;
#26877=CARTESIAN_POINT ( 'NONE',  ( -57.27248934188107654, -288.6512440413138165, -344.6864449927168152 ) ) ;
#26878=CARTESIAN_POINT ( 'NONE',  ( -22.23135365226562143, -284.4880363566454093, -197.8540352875978101 ) ) ;
#26880=CARTESIAN_POINT ( 'NONE',  ( -108.3343556861541970, -282.8723850060145537, -289.7844381861559100 ) ) ;
#26881=CARTESIAN_POINT ( 'NONE',  ( -42.76016990518110106, -287.3611652722732970, -344.2271534680248237 ) ) ;
#26882=CARTESIAN_POINT ( 'NONE',  ( -91.95026354765967369, -285.0589267341172786, -319.4211842818626224 ) ) ;
#26883=CARTESIAN_POINT ( 'NONE',  ( 37.14800832392594998, -273.6697087532749038, -279.5293646701454691 ) ) ;
#26884=CARTESIAN_POINT ( 'NONE',  ( 23.23796148366297487, -285.3290903211996579, -224.1169414945194944 ) ) ;
#26885=CARTESIAN_POINT ( 'NONE',  ( -110.9313838304562410, -298.7390324570658890, -255.8188038662694908 ) ) ;
#26886=CARTESIAN_POINT ( 'NONE',  ( -112.3210213468869938, -282.6287637666725914, -264.3684214495649485 ) ) ;
#26887=CARTESIAN_POINT ( 'NONE',  ( 33.33752256824769233, -282.2402889203216318, -251.1335982237621351 ) ) ;
#26888=CARTESIAN_POINT ( 'NONE',  ( -92.23606277049911739, -291.8342549185520056, -321.7842996216700726 ) ) ;
#26891=CARTESIAN_POINT ( 'NONE',  ( -11.52577693407175907, -296.6388007047333417, -341.4296799426973621 ) ) ;
#26892=CARTESIAN_POINT ( 'NONE',  ( -75.50204382171713746, -277.5434202744431218, -205.7352763166446437 ) ) ;
#26893=CARTESIAN_POINT ( 'NONE',  ( -109.0814529087638505, -294.7253750149093889, -287.7305967525836650 ) ) ;
#26894=CARTESIAN_POINT ( 'NONE',  ( -2.903275930910505398, -279.2021027020170436, -205.4219755186740883 ) ) ;
#26895=CARTESIAN_POINT ( 'NONE',  ( 27.91034656212066167, -273.1508603088242921, -234.4278689206720401 ) ) ;
#26896=CARTESIAN_POINT ( 'NONE',  ( 34.96537223064265731, -294.6941036798717732, -257.1409115309351705 ) ) ;
#26897=CARTESIAN_POINT ( 'NONE',  ( 21.31550574532285580, -290.6948066931273615, -317.0979686699210447 ) ) ;
#26898=CARTESIAN_POINT ( 'NONE',  ( -77.81814523701829955, -295.9987894828858543, -205.6744490061366264 ) ) ;
#26899=CARTESIAN_POINT ( 'NONE',  ( 34.50197405081497948, -291.4740911172476672, -245.4537650808617570 ) ) ;
#26900=CARTESIAN_POINT ( 'NONE',  ( -109.8605565985053971, -292.1448901237440055, -257.5641528542200263 ) ) ;
#26901=CARTESIAN_POINT ( 'NONE',  ( 120.8395553409046528, -299.5541904835127980, -195.3611179825600175 ) ) ;
#26902=CARTESIAN_POINT ( 'NONE',  ( -109.8615812104604998, -291.4871940426499464, -260.3170556970085840 ) ) ;
#26905=CARTESIAN_POINT ( 'NONE',  ( -113.6130288952681582, -291.8536350093470446, -262.6920504382006811 ) ) ;
#26906=CARTESIAN_POINT ( 'NONE',  ( 37.55107935066549629, -279.4598822186044913, -261.5674888522430024 ) ) ;
#26907=CARTESIAN_POINT ( 'NONE',  ( 33.94980566938370714, -293.3442674938572168, -254.6023236270237931 ) ) ;
#26908=CARTESIAN_POINT ( 'NONE',  ( 20.12868591505343119, -280.8571973516890807, -219.0952707735880267 ) ) ;
#26909=CARTESIAN_POINT ( 'NONE',  ( -50.09418622537307897, -282.8772141248481944, -346.3301839254096421 ) ) ;
#26910=CARTESIAN_POINT ( 'NONE',  ( 25.02364740037101143, -286.1121439429087445, -311.7438139391302343 ) ) ;
#26911=CARTESIAN_POINT ( 'NONE',  ( -67.07571345920861461, -281.5856783223593993, -338.3951675371041006 ) ) ;
#26913=CARTESIAN_POINT ( 'NONE',  ( 31.40531251692992853, -279.6019916771198268, -237.1252048540661121 ) ) ;
#26914=CARTESIAN_POINT ( 'NONE',  ( -29.48089718485516642, -285.0698438799033738, -194.0741578481965348 ) ) ;
#26916=CARTESIAN_POINT ( 'NONE',  ( -2.074870657405986751, -294.1273887602113177, -205.5186025678350461 ) ) ;
#26917=CARTESIAN_POINT ( 'NONE',  ( 23.99595064063498029, -276.3668564437114696, -224.7946951208070345 ) ) ;
#26918=CARTESIAN_POINT ( 'NONE',  ( -35.12124398369961398, -276.6902219015913147, -343.3484940236178886 ) ) ;
#26919=CARTESIAN_POINT ( 'NONE',  ( -112.5648884630178088, -290.5131509328750781, -286.8071491530723733 ) ) ;
#26920=CARTESIAN_POINT ( 'NONE',  ( -37.33931516258178362, -281.1319380449236291, -345.9339424150234663 ) ) ;
#26921=CARTESIAN_POINT ( 'NONE',  ( 19.53608827460852382, -291.9601006936595127, -224.2074999027515503 ) ) ;
#26922=CARTESIAN_POINT ( 'NONE',  ( -98.39563956292968783, -293.9586314611743774, -314.0079825295288742 ) ) ;
#26925=CARTESIAN_POINT ( 'NONE',  ( -2.404497430382225076, -292.0352512285432454, -206.1800939655338141 ) ) ;
#26926=CARTESIAN_POINT ( 'NONE',  ( -53.35057174420112602, -292.7666405000204577, -340.3538533559490702 ) ) ;
#26927=CARTESIAN_POINT ( 'NONE',  ( -112.3679711185133812, -295.8154061841117937, -254.0554609655942215 ) ) ;
#26928=CARTESIAN_POINT ( 'NONE',  ( -1.695295401843315952, -278.6590157914766337, -203.5057568470470244 ) ) ;
#26929=CARTESIAN_POINT ( 'NONE',  ( 25.93998426618589903, -288.2964805407460176, -227.3409005452003271 ) ) ;
#26930=CARTESIAN_POINT ( 'NONE',  ( -41.32080669932226158, -285.8340145623815829, -197.4571474487749470 ) ) ;
#26931=CARTESIAN_POINT ( 'NONE',  ( -67.06472314849371230, -278.9691491034104160, -337.7944158142855713 ) ) ;
#26932=CARTESIAN_POINT ( 'NONE',  ( -58.90699438193156112, -293.3526306158723855, -341.8228901694071737 ) ) ;
#26933=CARTESIAN_POINT ( 'NONE',  ( -89.19602700144785956, -297.5536340744403105, -323.2450780946124951 ) ) ;
#26934=CARTESIAN_POINT ( 'NONE',  ( -105.6428833645554874, -276.9896679005503302, -297.2326432929233988 ) ) ;
#26937=CARTESIAN_POINT ( 'NONE',  ( -95.56828596756385252, -295.5384795456581060, -320.7139629176973017 ) ) ;
#26938=CARTESIAN_POINT ( 'NONE',  ( -109.1472655586457563, -292.7266160176934591, -250.7326954000629939 ) ) ;
#26939=CARTESIAN_POINT ( 'NONE',  ( 202.4561393373856220, 292.0274278529104208, -53.99999999997706368 ) ) ;
#26940=CARTESIAN_POINT ( 'NONE',  ( 29.52164596457567569, -288.6021802054856948, -300.0364547155749051 ) ) ;
#26943=CARTESIAN_POINT ( 'NONE',  ( 18.99565118791591800, -279.8984700940976040, -218.2178244569315666 ) ) ;
#26944=CARTESIAN_POINT ( 'NONE',  ( -99.92071017042533754, -296.6097769036731506, -315.1406164243404646 ) ) ;
#26945=CARTESIAN_POINT ( 'NONE',  ( -97.35509213141698126, -289.3191698664828664, -224.0940724576813921 ) ) ;
#26946=CARTESIAN_POINT ( 'NONE',  ( -36.54515751558398051, -298.3951488193342811, -193.3822181063758592 ) ) ;
#26947=CARTESIAN_POINT ( 'NONE',  ( 34.92805796460896772, -293.7476428251430320, -259.9126945604775756 ) ) ;
#26951=CARTESIAN_POINT ( 'NONE',  ( -31.85710892106038372, -290.5043823095820699, -346.5225100210599862 ) ) ;
#26952=CARTESIAN_POINT ( 'NONE',  ( -111.2869819898779866, -281.4805209788416960, -234.7871824221999191 ) ) ;
#26954=CARTESIAN_POINT ( 'NONE',  ( 36.88879320862066891, -280.6483970606656726, -250.2326502778686290 ) ) ;
#26955=CARTESIAN_POINT ( 'NONE',  ( -60.57131821045653908, -287.7502956340750302, -199.2245361945525985 ) ) ;
#26956=CARTESIAN_POINT ( 'NONE',  ( 25.07436444961066258, -285.5388665922002929, -226.2608800461145790 ) ) ;
#26957=CARTESIAN_POINT ( 'NONE',  ( -94.29287010943507141, -271.2258015976106549, -221.7965970094414274 ) ) ;
#26958=CARTESIAN_POINT ( 'NONE',  ( -8.433762185400381028, -276.3535585208446719, -201.7084461572123359 ) ) ;
#26959=CARTESIAN_POINT ( 'NONE',  ( -95.39892191071538718, -289.2779651031976300, -223.7503861869165291 ) ) ;
#26960=CARTESIAN_POINT ( 'NONE',  ( -84.08539553021272184, -279.5468794929855676, -330.0543740339704755 ) ) ;
#26961=ORIENTED_EDGE ( 'NONE', *, *, #51060, .F. ) ;
#26962=CARTESIAN_POINT ( 'NONE',  ( -67.30628832385720273, -279.6479354901900365, -203.7808274495207570 ) ) ;
#26963=CARTESIAN_POINT ( 'NONE',  ( 2.766833846158528676, -279.9542100094539023, -209.1841064299111679 ) ) ;
#26964=CARTESIAN_POINT ( 'NONE',  ( 39.00817925293942068, -276.5343402955103329, -262.5979085935651938 ) ) ;
#26965=CARTESIAN_POINT ( 'NONE',  ( -105.8137324909532850, -277.7925123785902315, -235.8978731656794707 ) ) ;
#26966=CARTESIAN_POINT ( 'NONE',  ( 199.7521944962045666, 291.7792511365457813, -82.56829223883464408 ) ) ;
#26967=CARTESIAN_POINT ( 'NONE',  ( -106.6359884490323680, -273.9181512150559570, -237.3289848638757462 ) ) ;
#26968=CARTESIAN_POINT ( 'NONE',  ( -20.68810176410567081, -299.6820650060397497, -193.9463967560282640 ) ) ;
#26969=CARTESIAN_POINT ( 'NONE',  ( 31.98288692825981272, -284.4805209788416960, -303.7098442033569654 ) ) ;
#26972=CARTESIAN_POINT ( 'NONE',  ( 30.24142360882560965, -288.2507365597584794, -241.8264150553090133 ) ) ;
#26973=CARTESIAN_POINT ( 'NONE',  ( 33.11133244103795192, -289.6801019631970462, -298.9679176900412472 ) ) ;
#26974=CARTESIAN_POINT ( 'NONE',  ( -106.1312907718636751, -289.5717543808887626, -295.0974250455375341 ) ) ;
#26975=CARTESIAN_POINT ( 'NONE',  ( -86.06824191627872267, -283.2148303486321197, -329.9031286004266690 ) ) ;
#26976=CARTESIAN_POINT ( 'NONE',  ( 28.50428463181116356, -279.5030884062015275, -236.9198781703234999 ) ) ;
#26977=CARTESIAN_POINT ( 'NONE',  ( -82.24422209915924498, -287.2924405619603476, -211.2457308303927732 ) ) ;
#26978=CARTESIAN_POINT ( 'NONE',  ( 35.38470208894436553, -280.1875121436668223, -282.2597806675934748 ) ) ;
#26980=CARTESIAN_POINT ( 'NONE',  ( -101.2488366394426151, -280.3610249661507510, -234.0689510607662953 ) ) ;
#26981=CARTESIAN_POINT ( 'NONE',  ( -6.244744053618578761, -277.1245637039351664, -336.4881936594808849 ) ) ;
#26982=CARTESIAN_POINT ( 'NONE',  ( -107.3746178472144095, -288.9474663571093629, -301.5303129079152882 ) ) ;
#26984=CARTESIAN_POINT ( 'NONE',  ( -103.9056962709803713, -285.8562167720805860, -231.8704799858673482 ) ) ;
#26985=CARTESIAN_POINT ( 'NONE',  ( -58.46382961901134934, -283.8103215394305607, -344.3988831013352296 ) ) ;
#26986=CARTESIAN_POINT ( 'NONE',  ( 5.593803564284941743, -282.6187377573604635, -329.3996014248699566 ) ) ;
#26988=CARTESIAN_POINT ( 'NONE',  ( -87.84405725080166860, -293.2154311974926486, -213.8826494905186451 ) ) ;
#26990=CARTESIAN_POINT ( 'NONE',  ( -4.798605359621682886, -291.1566862305271570, -201.1206294100695402 ) ) ;
#26991=CARTESIAN_POINT ( 'NONE',  ( 34.35414921139504685, -274.4136814676367067, -255.3628606018893379 ) ) ;
#26992=CARTESIAN_POINT ( 'NONE',  ( -101.5477394236903450, -295.3424703599969234, -312.7764287083693944 ) ) ;
#26994=CARTESIAN_POINT ( 'NONE',  ( -96.33487913841184991, -288.4177170754038571, -314.5467917634023820 ) ) ;
#26995=CARTESIAN_POINT ( 'NONE',  ( 36.30600289774800871, -291.6899377816716310, -262.5164834725144374 ) ) ;
#26996=CARTESIAN_POINT ( 'NONE',  ( -72.53584868215146741, -290.7342172263004727, -334.7699870382133440 ) ) ;
#26998=CARTESIAN_POINT ( 'NONE',  ( -111.3814931968941693, -292.3987112909525194, -282.3239643039578937 ) ) ;
#26999=CARTESIAN_POINT ( 'NONE',  ( 35.97879999499883752, -291.3392100398112348, -253.7463668269542723 ) ) ;
#27000=CARTESIAN_POINT ( 'NONE',  ( 27.34847888445247932, -296.0606773808831349, -308.4115292890044771 ) ) ;
#27001=CARTESIAN_POINT ( 'NONE',  ( -54.82408830424453328, -286.7632512385069390, -199.1906170051136939 ) ) ;
#27002=CARTESIAN_POINT ( 'NONE',  ( -0.3392588022769228995, -296.5615698032382284, -335.8041264422155905 ) ) ;
#27003=CARTESIAN_POINT ( 'NONE',  ( 36.57402137300812939, -277.7193677872832041, -285.0196622779927225 ) ) ;
#27004=CARTESIAN_POINT ( 'NONE',  ( -37.24350971211693206, -297.2505260664353841, -193.5218439957791361 ) ) ;
#27005=CARTESIAN_POINT ( 'NONE',  ( -59.51970141286975036, -275.5831750314205237, -340.9735125801483946 ) ) ;
#27006=CARTESIAN_POINT ( 'NONE',  ( -1.246844991914348721, -278.6148118081109146, -205.2575417990964297 ) ) ;
#27007=CARTESIAN_POINT ( 'NONE',  ( -40.80897648240764397, -275.2127873590252989, -196.9960161790945961 ) ) ;
#27008=CARTESIAN_POINT ( 'NONE',  ( 34.17668587304616779, -273.7839170451136965, -243.4589478916424525 ) ) ;
#27009=CARTESIAN_POINT ( 'NONE',  ( -41.05090993925329457, -296.5249858741252638, -343.8694783810712465 ) ) ;
#27011=CARTESIAN_POINT ( 'NONE',  ( -110.3740837728159363, -297.4121711791267444, -266.0168498387822069 ) ) ;
#27013=CARTESIAN_POINT ( 'NONE',  ( 21.71883313833140505, -284.9321556821907961, -223.5403258825938337 ) ) ;
#27014=CARTESIAN_POINT ( 'NONE',  ( -89.24067963260355896, -273.1295864742683648, -219.0240365414788641 ) ) ;
#27015=CARTESIAN_POINT ( 'NONE',  ( 30.13156083459476164, -287.0704354751360938, -233.1511719122246120 ) ) ;
#27016=CARTESIAN_POINT ( 'NONE',  ( 0.7051482268294290146, -288.2263178266584873, -337.3405697443773761 ) ) ;
#27017=CARTESIAN_POINT ( 'NONE',  ( -106.8479408804492152, -298.1521704616210968, -299.6042945670899940 ) ) ;
#27018=CARTESIAN_POINT ( 'NONE',  ( -17.76481570027202039, -292.7989158339788105, -342.5883567483839443 ) ) ;
#27019=CARTESIAN_POINT ( 'NONE',  ( 21.47979334249457040, -281.4164219004883307, -319.7998753187028456 ) ) ;
#27020=CARTESIAN_POINT ( 'NONE',  ( -110.4683760289727132, -287.8380690714490129, -287.0191576251351080 ) ) ;
#27021=CARTESIAN_POINT ( 'NONE',  ( -23.74566243433469737, -278.2255832233853994, -196.5515232647989308 ) ) ;
#27022=CARTESIAN_POINT ( 'NONE',  ( -97.68405773378863444, -288.7678176850375280, -312.1675366423921218 ) ) ;
#27024=CARTESIAN_POINT ( 'NONE',  ( -98.19591294511941726, -287.9553087231412292, -314.1990631109609353 ) ) ;
#27025=CARTESIAN_POINT ( 'NONE',  ( -95.93654207537565526, -298.7768366597117051, -225.4731053042661131 ) ) ;
#27026=CARTESIAN_POINT ( 'NONE',  ( 33.76935068669640572, -282.6185675392887333, -242.2556625177731462 ) ) ;
#27027=CARTESIAN_POINT ( 'NONE',  ( -26.47972962276536890, -296.2075940571009482, -195.0095530692215391 ) ) ;
#27028=CARTESIAN_POINT ( 'NONE',  ( 34.33424141048760703, -281.3687042817164752, -256.4547656897550496 ) ) ;
#27029=CARTESIAN_POINT ( 'NONE',  ( -108.8893852687383088, -297.0814523879359399, -241.7585761403979063 ) ) ;
#27030=CARTESIAN_POINT ( 'NONE',  ( -91.56891983142160996, -274.6858094713000469, -220.5952624538230111 ) ) ;
#27031=CARTESIAN_POINT ( 'NONE',  ( 37.65808555574718497, -285.7543958104470221, -279.9648788667705048 ) ) ;
#27032=CARTESIAN_POINT ( 'NONE',  ( 11.66556568847853548, -282.7326330439566959, -213.5871050624455449 ) ) ;
#27033=CARTESIAN_POINT ( 'NONE',  ( -90.41092895989248746, -272.1989622165203286, -219.7672380726040160 ) ) ;
#27036=CARTESIAN_POINT ( 'NONE',  ( -110.2773358457840800, -286.7377079611017621, -254.4192920299765888 ) ) ;
#27038=CARTESIAN_POINT ( 'NONE',  ( -88.47809603358389552, -282.9094976428776249, -206.1857440867352693 ) ) ;
#27039=CARTESIAN_POINT ( 'NONE',  ( 18.77827521832830016, -275.4666970422026111, -322.8464224743636350 ) ) ;
#27040=CARTESIAN_POINT ( 'NONE',  ( -37.52297078781109718, -284.5746206262545570, -344.0667779758421716 ) ) ;
#27041=CARTESIAN_POINT ( 'NONE',  ( 35.62964301964243674, -277.0072732172582732, -259.2479396345030977 ) ) ;
#27042=CARTESIAN_POINT ( 'NONE',  ( -70.20015606914390105, -284.9018599522739805, -339.3604527272919427 ) ) ;
#27043=CARTESIAN_POINT ( 'NONE',  ( -53.79351812100647834, -282.0628097881499912, -341.9429800810540883 ) ) ;
#27044=CARTESIAN_POINT ( 'NONE',  ( 30.77885051945479944, -283.1388142576619771, -238.8585533059634542 ) ) ;
#27045=CARTESIAN_POINT ( 'NONE',  ( 21.84949606180241943, -275.0564338273549652, -221.1127444242365243 ) ) ;
#27046=CARTESIAN_POINT ( 'NONE',  ( 26.14576994433442181, -274.8102008817908199, -226.7677900761915453 ) ) ;
#27048=CARTESIAN_POINT ( 'NONE',  ( -39.71084415205695706, -297.0022590172003447, -344.7760879756850159 ) ) ;
#27049=CARTESIAN_POINT ( 'NONE',  ( 133.0872704186301405, -299.5541904835127980, -201.0153591320744226 ) ) ;
#27051=CARTESIAN_POINT ( 'NONE',  ( -74.02934795143775659, -293.6733790819649244, -336.7095634250213152 ) ) ;
#27052=CARTESIAN_POINT ( 'NONE',  ( 26.81779690022809604, -275.5377601327008392, -305.4175059622414210 ) ) ;
#27053=CARTESIAN_POINT ( 'NONE',  ( -9.264863866584025942, -299.4756024643253909, -193.6652131360563658 ) ) ;
#27054=CARTESIAN_POINT ( 'NONE',  ( -62.93401431314136829, -287.4746047551155925, -200.8585788520988729 ) ) ;
#27055=CARTESIAN_POINT ( 'NONE',  ( 25.15799781755510267, -295.6566403369897671, -314.1617265670072925 ) ) ;
#27056=CARTESIAN_POINT ( 'NONE',  ( 8.679908101217730376, -295.6420228036429307, -331.5985272475140277 ) ) ;
#27057=CARTESIAN_POINT ( 'NONE',  ( -105.2299404564854797, -292.9668639532366683, -238.8775468937512585 ) ) ;
#27058=CARTESIAN_POINT ( 'NONE',  ( 16.59809248660833703, -278.8207651292980245, -218.4167715059619468 ) ) ;
#27059=CARTESIAN_POINT ( 'NONE',  ( -111.4013365498536814, -280.5759484167172104, -262.3498738287158289 ) ) ;
#27060=CARTESIAN_POINT ( 'NONE',  ( -67.90843236900225577, -293.5363679146383333, -338.2499013958244518 ) ) ;
#27061=CARTESIAN_POINT ( 'NONE',  ( 1.481871720928115810, -284.3995048165134563, -335.4229020732794879 ) ) ;
#27062=CARTESIAN_POINT ( 'NONE',  ( -81.65454514863819213, -284.3528263942825447, -211.9607940207285708 ) ) ;
#27063=CARTESIAN_POINT ( 'NONE',  ( -20.24027634894776284, -109.4294513019383714, -361.8272583522734180 ) ) ;
#27065=CARTESIAN_POINT ( 'NONE',  ( -103.5028248555976802, -284.6374363640584306, -239.3415419039653784 ) ) ;
#27067=CARTESIAN_POINT ( 'NONE',  ( 37.37321837455115769, -282.4139734262460593, -253.0068341873516431 ) ) ;
#27068=CARTESIAN_POINT ( 'NONE',  ( -83.20715926477177504, -273.7368716614819277, -213.5416922123357892 ) ) ;
#27069=CARTESIAN_POINT ( 'NONE',  ( -70.87847623874073122, -284.4144237659661485, -201.4895464261220752 ) ) ;
#27070=CARTESIAN_POINT ( 'NONE',  ( -56.50952512321615728, -280.7523419835703749, -195.9731500756377898 ) ) ;
#27072=CARTESIAN_POINT ( 'NONE',  ( -95.60713845284749368, -279.4021525217668795, -319.6544608993764882 ) ) ;
#27073=CARTESIAN_POINT ( 'NONE',  ( 22.79040588354024166, -281.5607520303948945, -222.4085415732644719 ) ) ;
#27074=CARTESIAN_POINT ( 'NONE',  ( 30.89617123739170168, -273.2666405000204009, -285.9686137636504668 ) ) ;
#27075=CARTESIAN_POINT ( 'NONE',  ( 46.06605720673547211, 12.00925050775455105, -332.0840745435668282 ) ) ;
#27077=CARTESIAN_POINT ( 'NONE',  ( -31.21436617461464280, -276.1298694289623654, -195.7660872308242688 ) ) ;
#27078=CARTESIAN_POINT ( 'NONE',  ( 5.081724044709708288, -58.07489044105351184, -354.5077726519059524 ) ) ;
#27079=CARTESIAN_POINT ( 'NONE',  ( -72.89133565225273514, -277.5987852784263055, -204.7252267440417484 ) ) ;
#27080=CARTESIAN_POINT ( 'NONE',  ( 20.52401373771774473, -294.6391871028262130, -221.0915450451410891 ) ) ;
#27081=CARTESIAN_POINT ( 'NONE',  ( -109.2438962974729151, -295.7260717527908582, -283.6201532793220395 ) ) ;
#27082=CARTESIAN_POINT ( 'NONE',  ( -57.28100147874644676, -288.8102844577184101, -344.7260126453617772 ) ) ;
#27084=CARTESIAN_POINT ( 'NONE',  ( -66.71484145980906533, -294.0042132043214451, -340.9147396240794592 ) ) ;
#27085=CARTESIAN_POINT ( 'NONE',  ( 11.68051854302299297, -285.1456195826879139, -215.1266671553816821 ) ) ;
#27086=CARTESIAN_POINT ( 'NONE',  ( -75.63677188178273525, -293.3961697552185228, -206.7058659580672213 ) ) ;
#27087=CARTESIAN_POINT ( 'NONE',  ( -109.9107325604008878, -286.0206096022957354, -258.6632447618484889 ) ) ;
#27089=CARTESIAN_POINT ( 'NONE',  ( -68.24507237474850285, -292.5973546837572599, -200.0772997397733093 ) ) ;
#27090=CARTESIAN_POINT ( 'NONE',  ( 19.40380042737718824, -282.6953004464953096, -316.4018852143359481 ) ) ;
#27091=CARTESIAN_POINT ( 'NONE',  ( -99.69428786894694383, -294.7535877865786347, -314.9495132747550201 ) ) ;
#27092=CARTESIAN_POINT ( 'NONE',  ( -110.6247391956302408, -291.0620713887373654, -293.6380060135784902 ) ) ;
#27093=CARTESIAN_POINT ( 'NONE',  ( -114.3074426481026507, -291.0695130048759438, -268.3625722094486150 ) ) ;
#27094=CARTESIAN_POINT ( 'NONE',  ( 28.22869212883852086, -288.1534561859114092, -302.4473091519167838 ) ) ;
#27097=CARTESIAN_POINT ( 'NONE',  ( -58.48355652643064673, -297.1829074632005927, -343.1710502043929409 ) ) ;
#27098=CARTESIAN_POINT ( 'NONE',  ( -26.28145854419760141, -296.8727291153725787, -193.8566772683458055 ) ) ;
#27100=CARTESIAN_POINT ( 'NONE',  ( -39.69682902585414297, -279.0806313968635664, -197.1511409979437133 ) ) ;
#27102=CARTESIAN_POINT ( 'NONE',  ( 33.65918317144509331, -274.6810417403477231, -240.5856511379769245 ) ) ;
#27104=CARTESIAN_POINT ( 'NONE',  ( -101.8118574708835808, -295.5153437075560419, -234.6636872200012647 ) ) ;
#27105=CARTESIAN_POINT ( 'NONE',  ( 8.359146216502605142, -278.2799001800425458, -328.9270474524835777 ) ) ;
#27106=CARTESIAN_POINT ( 'NONE',  ( 24.84088220355097221, -273.1392364663823855, -229.8124813281596914 ) ) ;
#27107=CARTESIAN_POINT ( 'NONE',  ( -86.74598543921285909, -296.9628411107131569, -324.6413823225639703 ) ) ;
#27108=CARTESIAN_POINT ( 'NONE',  ( -95.00811062789185257, -296.9962205168547484, -315.6249133906281941 ) ) ;
#27109=DIRECTION ( 'NONE',  ( 0.000000000000000000, 0.000000000000000000, -1.000000000000000000 ) ) ;
#27110=CARTESIAN_POINT ( 'NONE',  ( -37.66491856410779349, -296.6562215843950980, -346.5733780863321840 ) ) ;
#27111=CARTESIAN_POINT ( 'NONE',  ( -67.41987226175098158, -295.6585651288866643, -201.4193128339187524 ) ) ;
#27112=CARTESIAN_POINT ( 'NONE',  ( -41.60706777165610504, -292.6485693250633062, -197.3338131666275785 ) ) ;
#27113=CARTESIAN_POINT ( 'NONE',  ( -71.34057051661984872, -274.4174295687763561, -201.4536754701578616 ) ) ;
#27114=CARTESIAN_POINT ( 'NONE',  ( -93.88098888094916106, -289.7900358237721434, -223.2385464290872505 ) ) ;
#27116=CARTESIAN_POINT ( 'NONE',  ( -52.53960631940750403, -274.3549741703365044, -194.8842391606416982 ) ) ;
#27117=CARTESIAN_POINT ( 'NONE',  ( -108.3185624601739931, -296.6584711917766413, -287.5711214357452263 ) ) ;
#27118=CARTESIAN_POINT ( 'NONE',  ( -73.00984370864296125, -281.5618258474715390, -203.9673435512872288 ) ) ;
#27119=CARTESIAN_POINT ( 'NONE',  ( 37.77371620120204909, -280.0541586373303744, -255.8362254300273833 ) ) ;
#27121=CARTESIAN_POINT ( 'NONE',  ( -91.26348299585882273, -277.1428869592384672, -325.2604526235271578 ) ) ;
#27122=CARTESIAN_POINT ( 'NONE',  ( -33.93048228879852246, -278.4942724223177493, -194.2375079162283669 ) ) ;
#27123=CARTESIAN_POINT ( 'NONE',  ( -2.506934465997397332, -280.5922660104716897, -336.9686815969719191 ) ) ;
#27124=CARTESIAN_POINT ( 'NONE',  ( -46.23211325318499121, -272.5118806592818146, -197.3108923092862597 ) ) ;
#27125=CARTESIAN_POINT ( 'NONE',  ( -51.49900481617321191, -279.2332408641801749, -344.0649843628651183 ) ) ;
#27128=CARTESIAN_POINT ( 'NONE',  ( -29.17248944189995541, -296.3929571019469336, -194.3768531707440559 ) ) ;
#27129=CARTESIAN_POINT ( 'NONE',  ( -11.15325247941416897, -292.3840816982365141, -197.8953764621370226 ) ) ;
#27130=CARTESIAN_POINT ( 'NONE',  ( 22.08466284731795426, -278.1820719640847415, -316.4095562690440033 ) ) ;
#27131=CARTESIAN_POINT ( 'NONE',  ( -1.947924874506630433, -272.5208028042094952, -204.2378896559987993 ) ) ;
#27133=CARTESIAN_POINT ( 'NONE',  ( -27.53431744379120261, -284.8487841724237910, -345.3343034640898850 ) ) ;
#27135=CARTESIAN_POINT ( 'NONE',  ( 34.53366031906455902, -285.8284808977682019, -291.8280710323473954 ) ) ;
#27137=CARTESIAN_POINT ( 'NONE',  ( 8.464066998315896484, -293.2040172695499223, -327.7758999392900137 ) ) ;
#27138=CARTESIAN_POINT ( 'NONE',  ( 29.93927130301597472, -285.2751941564156368, -238.9901702644280874 ) ) ;
#27140=CARTESIAN_POINT ( 'NONE',  ( -70.63416007385208673, -293.4910443560739282, -337.5668674673837018 ) ) ;
#27141=CARTESIAN_POINT ( 'NONE',  ( -62.95036322880340407, -284.2045262477641927, -198.4799373703612275 ) ) ;
#27142=CARTESIAN_POINT ( 'NONE',  ( -107.2086285578391198, -280.4666061661100684, -246.4332172486349180 ) ) ;
#27143=CARTESIAN_POINT ( 'NONE',  ( 33.48639945661435036, -288.3829295627783722, -241.0440397873470033 ) ) ;
#27144=CARTESIAN_POINT ( 'NONE',  ( 23.79003188677680569, -279.1842669142483828, -225.2292516735357424 ) ) ;
#27145=CARTESIAN_POINT ( 'NONE',  ( 35.45189963851188963, -287.6328880002740220, -276.4813352767075116 ) ) ;
#27146=CARTESIAN_POINT ( 'NONE',  ( -16.77428359631433352, -281.7483690541880605, -199.7045097072040392 ) ) ;
#27147=CARTESIAN_POINT ( 'NONE',  ( 21.45265491560540383, -281.7455858576137757, -226.7989577140384085 ) ) ;
#27148=CARTESIAN_POINT ( 'NONE',  ( -0.5419497714532174326, -288.5185094191756434, -204.5878571854532595 ) ) ;
#27150=CARTESIAN_POINT ( 'NONE',  ( -60.14606401076753883, -297.5979643126483438, -196.7599576213100363 ) ) ;
#27151=CARTESIAN_POINT ( 'NONE',  ( -109.3049033929112994, -292.2736117586874798, -290.3792184289671923 ) ) ;
#27153=CARTESIAN_POINT ( 'NONE',  ( 40.64545035920995986, -295.8376638359844719, -252.5284128619064461 ) ) ;
#27155=CARTESIAN_POINT ( 'NONE',  ( -82.45883904449129886, -271.4379707684648224, -210.1755097386434272 ) ) ;
#27157=CARTESIAN_POINT ( 'NONE',  ( -22.27585476842065759, -293.2621707371192770, -345.0569057958156804 ) ) ;
#27158=CARTESIAN_POINT ( 'NONE',  ( -103.2934757685224838, -272.3265897374299129, -238.8292934603810522 ) ) ;
#27159=CARTESIAN_POINT ( 'NONE',  ( -89.13473193361593871, -291.3171703720088885, -322.7842961399212527 ) ) ;
#27160=CARTESIAN_POINT ( 'NONE',  ( 36.71706668637780524, -283.3245770910309602, -271.3046127958364764 ) ) ;
#27161=CARTESIAN_POINT ( 'NONE',  ( -40.29765243386989226, -290.5138626856029873, -346.7276762444335532 ) ) ;
#27162=CARTESIAN_POINT ( 'NONE',  ( -96.89557629440854214, -291.2191001342065988, -318.4092038235149857 ) ) ;
#27163=CARTESIAN_POINT ( 'NONE',  ( 3.515788104972966899, -288.6018247231436362, -207.4670300057369161 ) ) ;
#27164=CARTESIAN_POINT ( 'NONE',  ( -82.24057840012150677, -279.6247353396032622, -207.8064160457798550 ) ) ;
#27165=CARTESIAN_POINT ( 'NONE',  ( 14.47311252195236975, -292.4098536690461287, -325.3569304242728322 ) ) ;
#27166=CARTESIAN_POINT ( 'NONE',  ( -67.88330470271029071, -283.2754385115422906, -341.0449944645973233 ) ) ;
#27167=CARTESIAN_POINT ( 'NONE',  ( 24.06091381193657242, -276.8417265180103186, -228.6180145796591319 ) ) ;
#27168=CARTESIAN_POINT ( 'NONE',  ( -37.30987171927208124, -279.5519495502701375, -340.3611179825599606 ) ) ;
#27170=CARTESIAN_POINT ( 'NONE',  ( 12.02900407612087719, -274.6163907632532073, -328.1236281235106276 ) ) ;
#27172=CARTESIAN_POINT ( 'NONE',  ( 34.76328193353419493, -281.2151209592579448, -282.1450054410386201 ) ) ;
#27173=CARTESIAN_POINT ( 'NONE',  ( -41.34825205859600317, -278.3065845108381495, -346.8723388795421556 ) ) ;
#27175=CARTESIAN_POINT ( 'NONE',  ( -43.54030390261068106, -275.2875319754132306, -197.0787814104780011 ) ) ;
#27176=CARTESIAN_POINT ( 'NONE',  ( -111.4907914037313219, -283.8626972706166498, -250.2935761317594086 ) ) ;
#27177=CARTESIAN_POINT ( 'NONE',  ( -44.41911495301716428, -293.7216902271754861, -196.6354178582184318 ) ) ;
#27178=CARTESIAN_POINT ( 'NONE',  ( -4.192740137663658828, -276.0819946351367093, -201.7349058634811172 ) ) ;
#27179=CARTESIAN_POINT ( 'NONE',  ( -76.19680184020130298, -274.8597966351502464, -204.3940593153448333 ) ) ;
#27181=CARTESIAN_POINT ( 'NONE',  ( 35.60182152929297672, -275.4376259677823100, -274.3147464286044510 ) ) ;
#27182=CARTESIAN_POINT ( 'NONE',  ( -109.2274080316977773, -298.8206270627312620, -249.5651225237248525 ) ) ;
#27183=CARTESIAN_POINT ( 'NONE',  ( -49.69982063282382256, -283.8941529116401625, -196.5024668465094067 ) ) ;
#27184=CARTESIAN_POINT ( 'NONE',  ( 37.06324037213543221, -292.9711000339918883, -250.5707191875494857 ) ) ;
#27185=CARTESIAN_POINT ( 'NONE',  ( 37.34412841002156824, -273.5887231500738039, -271.6377031581768051 ) ) ;
#27186=CARTESIAN_POINT ( 'NONE',  ( 38.29904551428222703, -289.2741106656858960, -280.0015450561255648 ) ) ;
#27187=CARTESIAN_POINT ( 'NONE',  ( -107.2510278158380004, -289.1792097511361703, -292.5952010055052028 ) ) ;
#27189=CARTESIAN_POINT ( 'NONE',  ( -22.29194152094668624, -290.8158412550358207, -195.3931809736681089 ) ) ;
#27190=CARTESIAN_POINT ( 'NONE',  ( -108.7303444997062769, -290.4213577064709852, -255.0069999143981931 ) ) ;
#27192=CARTESIAN_POINT ( 'NONE',  ( 37.52619538189749449, -288.8412901908744743, -287.0431135365123509 ) ) ;
#27193=CARTESIAN_POINT ( 'NONE',  ( -72.14352144196793404, -279.9115849072436504, -206.1667200956572401 ) ) ;
#27194=CARTESIAN_POINT ( 'NONE',  ( -37.70138334217815412, -293.9768556387269314, -347.0641895681428650 ) ) ;
#27195=CARTESIAN_POINT ( 'NONE',  ( -23.81200429218027281, -286.8719398440842951, -194.6084923785239482 ) ) ;
#27197=CARTESIAN_POINT ( 'NONE',  ( -65.87347006701266139, -286.0222306590572430, -198.8509363197336199 ) ) ;
#27198=CARTESIAN_POINT ( 'NONE',  ( 1.116050935498282159, -282.8569347567111549, -332.4934169854815877 ) ) ;
#27199=CARTESIAN_POINT ( 'NONE',  ( -113.8401055986460477, -273.8937930856225194, -270.3782002851730226 ) ) ;
#27200=CARTESIAN_POINT ( 'NONE',  ( -14.23015497029708598, -91.07820911423134191, -358.7444012829247413 ) ) ;
#27201=CARTESIAN_POINT ( 'NONE',  ( 159.6170603531574841, 218.6245907200500938, -202.5626340042458082 ) ) ;
#27202=CARTESIAN_POINT ( 'NONE',  ( 33.74099093003696481, -274.9779143230453542, -287.7301175321651385 ) ) ;
#27203=CARTESIAN_POINT ( 'NONE',  ( 30.46595282356512868, -274.0990319840454958, -242.3647336413309006 ) ) ;
#27204=CARTESIAN_POINT ( 'NONE',  ( -111.1581219643938994, -295.7869338039098466, -292.1023643087694381 ) ) ;
#27205=CARTESIAN_POINT ( 'NONE',  ( -29.53615242528336537, -125.4933017954314209, -361.0433250153028553 ) ) ;
#27206=CARTESIAN_POINT ( 'NONE',  ( 32.11245255324794812, -273.8224313796083038, -238.1503406651623038 ) ) ;
#27207=CARTESIAN_POINT ( 'NONE',  ( -110.8952709848931306, -274.4194697368468496, -262.1242358750587300 ) ) ;
#27208=CARTESIAN_POINT ( 'NONE',  ( -84.03645773215937709, -292.4722694911574763, -213.8471755882974890 ) ) ;
#27210=CARTESIAN_POINT ( 'NONE',  ( -114.1305156203026030, -297.4668807950995415, -272.4753099720512068 ) ) ;
#27211=CARTESIAN_POINT ( 'NONE',  ( 35.33496714404230232, -287.9457882853840829, -262.8717604799663263 ) ) ;
#27212=CARTESIAN_POINT ( 'NONE',  ( -32.01347938135889848, -295.7894003584659117, -347.0279088065643691 ) ) ;
#27213=CARTESIAN_POINT ( 'NONE',  ( -97.35549281811060496, -296.3986872176711813, -318.5262453155505114 ) ) ;
#27214=CARTESIAN_POINT ( 'NONE',  ( 10.92921582374588496, -292.9085720158423101, -215.5312836712909643 ) ) ;
#27216=CARTESIAN_POINT ( 'NONE',  ( 32.37527916553901264, -277.0931546752253212, -241.0909381586193092 ) ) ;
#27217=EDGE_CURVE ( 'NONE', #34864, #58191, #66908, .T. ) ;
#27219=CARTESIAN_POINT ( 'NONE',  ( 36.54238063936777081, -280.7899038512508127, -248.8506603716031975 ) ) ;
#27220=CARTESIAN_POINT ( 'NONE',  ( -76.47144089843956749, -278.5305240449147846, -332.3261004382662236 ) ) ;
#27221=CARTESIAN_POINT ( 'NONE',  ( -0.5559044195958554591, -276.2941455033346756, -203.8573833218385118 ) ) ;
#27222=CARTESIAN_POINT ( 'NONE',  ( -41.32330150027915039, -275.1221310374358495, -345.6239857958984203 ) ) ;
#27223=CARTESIAN_POINT ( 'NONE',  ( -106.8062448494982135, -297.5072849462307545, -247.4284569389462831 ) ) ;
#27224=CARTESIAN_POINT ( 'NONE',  ( -96.89586621137789280, -294.5265235765434682, -313.6108207982694580 ) ) ;
#27226=CARTESIAN_POINT ( 'NONE',  ( 34.26484624583969918, -281.6857926547419879, -242.0727197365910115 ) ) ;
#27227=CARTESIAN_POINT ( 'NONE',  ( 11.74927274661883203, -276.5146099098660670, -324.4581901128391337 ) ) ;
#27228=CARTESIAN_POINT ( 'NONE',  ( 18.00638613757957884, -285.5093948314013801, -217.4653093328933835 ) ) ;
#27229=CARTESIAN_POINT ( 'NONE',  ( -48.71827311485052547, -299.9079007227234683, -196.0079738450369575 ) ) ;
#27230=CARTESIAN_POINT ( 'NONE',  ( 82.61707336526248469, -302.0539871969763226, -195.3101965168185075 ) ) ;
#27231=CARTESIAN_POINT ( 'NONE',  ( 20.47879813962316220, -287.3794791383505185, -315.2076369955311748 ) ) ;
#27232=CARTESIAN_POINT ( 'NONE',  ( -43.81772289878191629, -278.2091841065776521, -196.5807140211692285 ) ) ;
#27233=CARTESIAN_POINT ( 'NONE',  ( -77.12526444794451663, -278.0825939376779274, -208.3920389536815776 ) ) ;
#27234=CARTESIAN_POINT ( 'NONE',  ( -103.0536698178278385, -282.1633308060364698, -305.4459008541170988 ) ) ;
#27236=CARTESIAN_POINT ( 'NONE',  ( 12.04145225774467320, -288.7384753318011690, -213.8455216671241885 ) ) ;
#27237=CARTESIAN_POINT ( 'NONE',  ( 17.74334282199198398, -277.4462668281370838, -318.8854290802125320 ) ) ;
#27239=CARTESIAN_POINT ( 'NONE',  ( 0.6640562742306593824, -294.5586054158831075, -205.6445027228300830 ) ) ;
#27240=CARTESIAN_POINT ( 'NONE',  ( -97.14544960480280622, -276.1570363177626746, -317.2384639609127817 ) ) ;
#27241=AXIS2_PLACEMENT_3D ( 'NONE', #41305, #92443, #56015 ) ;
#27242=CARTESIAN_POINT ( 'NONE',  ( 33.99456047768848066, -276.4146899477607917, -286.3877439569877197 ) ) ;
#27243=CARTESIAN_POINT ( 'NONE',  ( 31.88760362947346039, -283.9355731600895183, -299.7743803571923422 ) ) ;
#27245=CARTESIAN_POINT ( 'NONE',  ( -111.9345162805996239, -292.3187177920996760, -282.4120921047509682 ) ) ;
#27247=CARTESIAN_POINT ( 'NONE',  ( -71.47367798673904815, -293.5027394604568372, -337.1586007794692819 ) ) ;
#27248=LINE ( 'NONE', #11629, #81422 ) ;
#27249=CARTESIAN_POINT ( 'NONE',  ( 9.814248056467786085, -273.4018467065816367, -213.9246120920402063 ) ) ;
#27250=CARTESIAN_POINT ( 'NONE',  ( 20.31995916252685674, -291.0410855286802416, -223.5863414245100387 ) ) ;
#27253=CARTESIAN_POINT ( 'NONE',  ( -112.2406604538473687, -289.2170132661147477, -255.7036377136570593 ) ) ;
#27254=CARTESIAN_POINT ( 'NONE',  ( -107.7429726196183566, -285.8620313682378651, -292.4993484210141901 ) ) ;
#27255=CARTESIAN_POINT ( 'NONE',  ( 33.09447819934654689, -286.1603862431920788, -299.0093903638906454 ) ) ;
#27256=CARTESIAN_POINT ( 'NONE',  ( -107.5425581094592786, -285.6872034938801335, -292.4340529031632627 ) ) ;
#27257=CARTESIAN_POINT ( 'NONE',  ( -93.38537246701778827, -286.0213424944082021, -223.3323127861600597 ) ) ;
#27258=CARTESIAN_POINT ( 'NONE',  ( -66.40487667731842691, -293.6533666926130195, -200.8360248634611196 ) ) ;
#27259=CARTESIAN_POINT ( 'NONE',  ( -5.906575967852359277, -274.7219908507835271, -339.0717224811123174 ) ) ;
#27260=CARTESIAN_POINT ( 'NONE',  ( 5.862923049857116986, -276.8169398349917856, -334.0722224111300420 ) ) ;
#27261=CARTESIAN_POINT ( 'NONE',  ( -98.71519760985064806, -288.0364577609849448, -314.4583219707833450 ) ) ;
#27262=CARTESIAN_POINT ( 'NONE',  ( -51.31261788592143347, -277.2260537685583586, -346.0830663000965615 ) ) ;
#27263=CARTESIAN_POINT ( 'NONE',  ( -102.9001396388044611, -298.0555785965820519, -306.0533833755586670 ) ) ;
#27266=CARTESIAN_POINT ( 'NONE',  ( -108.8414158629337720, -283.4603991874049029, -253.3059686449774972 ) ) ;
#27267=CARTESIAN_POINT ( 'NONE',  ( -107.7203582892381348, -276.8900631815772613, -244.2913449617409185 ) ) ;
#27269=CARTESIAN_POINT ( 'NONE',  ( 36.56237143450444194, -274.2719402145314689, -289.3583799184990539 ) ) ;
#27270=CARTESIAN_POINT ( 'NONE',  ( -66.85140617073518854, -276.7979650304584425, -337.2421311158539652 ) ) ;
#27271=CARTESIAN_POINT ( 'NONE',  ( -45.14508731213439319, -296.6727513510831500, -343.6910946173409798 ) ) ;
#27272=CARTESIAN_POINT ( 'NONE',  ( 12.80049110095817433, -279.6532969102798347, -212.3330802105268447 ) ) ;
#27273=CARTESIAN_POINT ( 'NONE',  ( -36.98239379526970794, -295.9887657759894068, -343.6079961080988028 ) ) ;
#27274=CARTESIAN_POINT ( 'NONE',  ( -66.71949139904042170, -296.7442169117479693, -341.0168837673675171 ) ) ;
#27275=CARTESIAN_POINT ( 'NONE',  ( -90.04439469925162598, -297.1151031139099246, -219.7771372823663114 ) ) ;
#27276=CARTESIAN_POINT ( 'NONE',  ( -63.52210236830130441, -293.7111094891626522, -200.0789211828130476 ) ) ;
#27277=CARTESIAN_POINT ( 'NONE',  ( -71.06814580863060371, -285.7859574561193767, -201.1402622648361103 ) ) ;
#27278=CARTESIAN_POINT ( 'NONE',  ( 35.40663502596412826, -273.4198770511666226, -249.0119162494369220 ) ) ;
#27279=CARTESIAN_POINT ( 'NONE',  ( 12.41421110037587461, -288.2143355142272867, -329.1263228431822085 ) ) ;
#27280=CARTESIAN_POINT ( 'NONE',  ( -30.12797466507436539, -282.1236338135403230, -196.0142116669283041 ) ) ;
#27281=EDGE_CURVE ( 'NONE', #36646, #19844, #8821, .T. ) ;
#27282=CARTESIAN_POINT ( 'NONE',  ( -105.7805722437432223, -283.9578323582138637, -244.2933365036481632 ) ) ;
#27283=CARTESIAN_POINT ( 'NONE',  ( -109.9912506668829053, -288.3120511554026848, -289.0416670026615407 ) ) ;
#27284=CARTESIAN_POINT ( 'NONE',  ( -101.7183354143585632, -264.3591293023451385, -316.7762957234928649 ) ) ;
#27285=CARTESIAN_POINT ( 'NONE',  ( -52.09524032839020435, -285.3658030966421393, -198.8046962370723918 ) ) ;
#27287=CARTESIAN_POINT ( 'NONE',  ( 35.39002270344933976, -282.8054892677800467, -295.0807508349498676 ) ) ;
#27288=CARTESIAN_POINT ( 'NONE',  ( -99.00839927858632450, -290.2207869571089986, -224.6221640959064700 ) ) ;
#27289=CARTESIAN_POINT ( 'NONE',  ( -108.9776323251525270, -279.8189887089838521, -296.4909942747548257 ) ) ;
#27290=CARTESIAN_POINT ( 'NONE',  ( -71.03261470167893776, -280.9319777028852059, -201.6718135009071773 ) ) ;
#27291=CARTESIAN_POINT ( 'NONE',  ( 17.60345822387882464, -282.0712386883000704, -318.4238850502009655 ) ) ;
#27292=CARTESIAN_POINT ( 'NONE',  ( 37.70037354433792132, -277.5681354000283250, -271.5930769435605043 ) ) ;
#27293=CARTESIAN_POINT ( 'NONE',  ( -0.7061756425740647325, -294.5792951268875299, -338.1022046013854379 ) ) ;
#27294=CARTESIAN_POINT ( 'NONE',  ( -110.8020079200934305, -288.4013858065329714, -283.6061164272788915 ) ) ;
#27295=CARTESIAN_POINT ( 'NONE',  ( -109.6701288752704357, -295.3154890322894062, -282.3120371511369058 ) ) ;
#27298=CARTESIAN_POINT ( 'NONE',  ( 23.78085754748449077, -284.0530328643782809, -312.8504947958872435 ) ) ;
#27299=CARTESIAN_POINT ( 'NONE',  ( -106.0085204806748322, -295.8863136437994967, -295.3484049681551369 ) ) ;
#27300=CARTESIAN_POINT ( 'NONE',  ( 38.91721238381406778, -294.5236544807613086, -261.7469259622861273 ) ) ;
#27301=CARTESIAN_POINT ( 'NONE',  ( -66.59275217290401372, -284.0971014425639964, -337.3692488707681605 ) ) ;
#27302=CARTESIAN_POINT ( 'NONE',  ( 36.36333780702232588, -274.3388925976531141, -248.7186136124020095 ) ) ;
#27303=CARTESIAN_POINT ( 'NONE',  ( -108.2763090439945017, -291.5817165116959586, -240.6694685799345450 ) ) ;
#27304=CARTESIAN_POINT ( 'NONE',  ( -65.39758372173835710, -283.8288876396491673, -199.9684111732740632 ) ) ;
#27306=CARTESIAN_POINT ( 'NONE',  ( -85.14822228928255754, -290.0247389172650401, -330.7638640423928109 ) ) ;
#27307=CARTESIAN_POINT ( 'NONE',  ( 30.50640403082802266, -288.2481497407778761, -297.4923682335670492 ) ) ;
#27310=CARTESIAN_POINT ( 'NONE',  ( 167.4109119493085700, 229.8605661533808870, -189.8721647499563687 ) ) ;
#27312=CARTESIAN_POINT ( 'NONE',  ( -21.84768608329982342, -284.3771770459457571, -345.0782062535183741 ) ) ;
#27313=CARTESIAN_POINT ( 'NONE',  ( -4.829096099716524648, -280.1237833571632336, -337.9475929042657754 ) ) ;
#27315=CARTESIAN_POINT ( 'NONE',  ( 30.61595329125420761, -280.8391301712606491, -297.8562705483535638 ) ) ;
#27316=CARTESIAN_POINT ( 'NONE',  ( 12.68765748498152668, -276.0430211412867152, -328.8658841838119429 ) ) ;
#27317=CARTESIAN_POINT ( 'NONE',  ( -95.87140642681021063, -279.9096711071192090, -317.0109887043710160 ) ) ;
#27318=CARTESIAN_POINT ( 'NONE',  ( 194.9847507448477586, 275.9312710741783690, -124.5726050330940495 ) ) ;
#27319=CARTESIAN_POINT ( 'NONE',  ( 16.81837667705199024, -279.3792732367631970, -216.3861421213827896 ) ) ;
#27320=CARTESIAN_POINT ( 'NONE',  ( -86.79746320437757845, -283.3808451009110172, -214.3816419668695801 ) ) ;
#27321=CARTESIAN_POINT ( 'NONE',  ( -93.88237814915559909, -297.6140871058700554, -321.1458961067387463 ) ) ;
#27322=CARTESIAN_POINT ( 'NONE',  ( 14.36425850722171305, -294.7935999725800116, -322.0508823860793655 ) ) ;
#27324=CARTESIAN_POINT ( 'NONE',  ( -103.2953156199358773, -288.8005705447496894, -302.7858628561513683 ) ) ;
#27325=CARTESIAN_POINT ( 'NONE',  ( -31.27638830350270993, -274.7782450094238129, -193.6893597177242725 ) ) ;
#27326=CARTESIAN_POINT ( 'NONE',  ( -63.30672211539041427, -273.7042447018218922, -202.1214005255021391 ) ) ;
#27328=CARTESIAN_POINT ( 'NONE',  ( -0.1831253113849828362, -273.4547914905875245, -203.2586824619305332 ) ) ;
#27332=CARTESIAN_POINT ( 'NONE',  ( 24.39816595799696941, -283.1774308882137916, -309.9818599623097839 ) ) ;
#27333=CARTESIAN_POINT ( 'NONE',  ( -92.35579478825694366, -281.0391018675192640, -217.8700442863209901 ) ) ;
#27334=CARTESIAN_POINT ( 'NONE',  ( -109.8434773210250626, -283.7468500849336692, -260.0218359929064604 ) ) ;
#27335=CARTESIAN_POINT ( 'NONE',  ( -30.16618188883983009, -282.0041768253495320, -196.4223111558342225 ) ) ;
#27336=CARTESIAN_POINT ( 'NONE',  ( -11.02434954015732949, -275.1826137930383993, -339.1950108740455789 ) ) ;
#27339=CARTESIAN_POINT ( 'NONE',  ( -91.20852860431287468, -278.5968984351251265, -325.2309066167078981 ) ) ;
#27343=CARTESIAN_POINT ( 'NONE',  ( -37.28952445085584344, -285.0313527085119745, -345.7290907686743822 ) ) ;
#27344=CARTESIAN_POINT ( 'NONE',  ( -3.552610916742571234, -291.7073486354183842, -205.4696765001656615 ) ) ;
#27346=CARTESIAN_POINT ( 'NONE',  ( -60.00515845156854766, -288.6869560250977997, -343.8436359249863017 ) ) ;
#27347=CARTESIAN_POINT ( 'NONE',  ( -74.03885036147005394, -283.7973853105481794, -206.0712863698774697 ) ) ;
#27348=CARTESIAN_POINT ( 'NONE',  ( -98.58748373413178001, -283.6886951472571923, -229.5649305666050566 ) ) ;
#27349=CARTESIAN_POINT ( 'NONE',  ( -91.34730427840381140, -288.0730640359070094, -321.0459539607400075 ) ) ;
#27350=CARTESIAN_POINT ( 'NONE',  ( -71.58058375418737285, -284.7202224335170513, -335.2828351021660183 ) ) ;
#27351=CARTESIAN_POINT ( 'NONE',  ( 36.21573023247668033, -273.7399587408131083, -285.0002808901811591 ) ) ;
#27352=CARTESIAN_POINT ( 'NONE',  ( 36.60546808372873784, -285.7195202817657105, -251.9693608252536876 ) ) ;
#27353=CARTESIAN_POINT ( 'NONE',  ( -111.6245334400059050, -298.6863644333126899, -259.9209482428871638 ) ) ;
#27354=CARTESIAN_POINT ( 'NONE',  ( -77.52046640878283768, -283.5141286249710220, -206.8339964871320831 ) ) ;
#27355=CARTESIAN_POINT ( 'NONE',  ( 15.42060562452119399, -281.7617032878529812, -219.4994397253662441 ) ) ;
#27356=CARTESIAN_POINT ( 'NONE',  ( 33.12643481780811072, -289.2135120760518703, -244.2025556733286749 ) ) ;
#27359=CARTESIAN_POINT ( 'NONE',  ( -0.1466359448418213252, -296.4815763022608053, -336.1471449682514390 ) ) ;
#27360=CARTESIAN_POINT ( 'NONE',  ( -94.60106717679414601, -277.2222716827536146, -221.9020741588640249 ) ) ;
#27361=CARTESIAN_POINT ( 'NONE',  ( -112.1577026689060972, -289.9688221063344713, -252.8475636552739445 ) ) ;
#27362=CARTESIAN_POINT ( 'NONE',  ( 8.711667836346627780, -292.8090281831858306, -328.0941692137078576 ) ) ;
#27363=CARTESIAN_POINT ( 'NONE',  ( -16.76772230498805882, -279.0083639460441418, -199.8064943679413545 ) ) ;
#27364=CARTESIAN_POINT ( 'NONE',  ( -111.0041586080609335, -270.7753642946829586, -259.2785438180432607 ) ) ;
#27365=CARTESIAN_POINT ( 'NONE',  ( 4.772621072075070359, -293.9490609137965862, -210.0689550756791562 ) ) ;
#27366=CARTESIAN_POINT ( 'NONE',  ( -69.85430415644619018, -297.9805209788416391, -337.9475929042657754 ) ) ;
#27367=CARTESIAN_POINT ( 'NONE',  ( -91.13293395096499694, -295.7842898866273913, -216.2389329227558505 ) ) ;
#27368=CARTESIAN_POINT ( 'NONE',  ( -50.87842608446878501, -290.8279796968201936, -342.9612582092462389 ) ) ;
#27369=CARTESIAN_POINT ( 'NONE',  ( 14.75988629442987765, -291.0134833856989189, -214.9770199582285670 ) ) ;
#27370=CARTESIAN_POINT ( 'NONE',  ( -107.1358418708726390, -292.2847520119598244, -247.0340372542501939 ) ) ;
#27372=CARTESIAN_POINT ( 'NONE',  ( -108.8705926296952384, -291.5572875698862276, -254.9916916755754528 ) ) ;
#27374=CARTESIAN_POINT ( 'NONE',  ( -108.4242666544780036, -291.3929707092885337, -298.9141818055691715 ) ) ;
#27375=CARTESIAN_POINT ( 'NONE',  ( 37.97503265957070795, -279.6030249995276336, -272.7687230323354015 ) ) ;
#27376=CARTESIAN_POINT ( 'NONE',  ( 23.34124622615589217, -292.9886269204886275, -229.7830448177489302 ) ) ;
#27377=CARTESIAN_POINT ( 'NONE',  ( -41.00839511846569962, -280.0072384461698221, -193.4352749524908859 ) ) ;
#27378=AXIS2_PLACEMENT_3D ( 'NONE', #23323, #2008, #67355 ) ;
#27379=CARTESIAN_POINT ( 'NONE',  ( -31.64208975497111709, -282.6488075958485524, -347.1419453093952256 ) ) ;
#27380=CARTESIAN_POINT ( 'NONE',  ( -69.57004763612914644, -287.4772168838541688, -337.8989743899766722 ) ) ;
#27381=CARTESIAN_POINT ( 'NONE',  ( 28.89402431627868495, -279.2428427415923124, -236.7255172946338178 ) ) ;
#27382=CARTESIAN_POINT ( 'NONE',  ( -15.95863829356263963, -284.3283997290398020, -198.4199873560102674 ) ) ;
#27383=CARTESIAN_POINT ( 'NONE',  ( 25.71866934945004601, -279.4591717714094443, -227.3026520576797793 ) ) ;
#27384=CARTESIAN_POINT ( 'NONE',  ( -26.65054086944309830, -285.1053071215373507, -194.3658049844564459 ) ) ;
#27386=CARTESIAN_POINT ( 'NONE',  ( 11.44455111512501588, -294.3417896529086875, -214.9183819441529693 ) ) ;
#27387=CARTESIAN_POINT ( 'NONE',  ( 25.64846991934734177, -276.4018962778529271, -227.0846712990225171 ) ) ;
#27388=CARTESIAN_POINT ( 'NONE',  ( -109.3076459926786583, -278.0547752691741721, -282.8039674619773791 ) ) ;
#27389=CARTESIAN_POINT ( 'NONE',  ( -107.7305083301197755, -290.3190013718808018, -301.7078813829190835 ) ) ;
#27390=CARTESIAN_POINT ( 'NONE',  ( -83.03226933975948043, -281.7513958574232902, -330.6073059821854372 ) ) ;
#27391=CARTESIAN_POINT ( 'NONE',  ( -108.3336134309491001, -289.8481472968634876, -252.3224674822463385 ) ) ;
#27392=CARTESIAN_POINT ( 'NONE',  ( -91.27690388316308656, -293.8190723161891356, -322.4763215629811270 ) ) ;
#27395=CARTESIAN_POINT ( 'NONE',  ( -30.79522088293225579, -291.6447872699930031, -197.5934599801285003 ) ) ;
#27397=CARTESIAN_POINT ( 'NONE',  ( -102.0172624299487154, -270.4809262143062369, -239.1787733560258289 ) ) ;
#27398=CARTESIAN_POINT ( 'NONE',  ( -113.5397675098091952, -295.7276931348159792, -261.0511910224050212 ) ) ;
#27399=CARTESIAN_POINT ( 'NONE',  ( 38.40674090728612811, -279.6507178174103387, -267.1340045153355049 ) ) ;
#27402=CARTESIAN_POINT ( 'NONE',  ( -113.8342913009046100, -285.9077191078187639, -267.1519065369233203 ) ) ;
#27403=CARTESIAN_POINT ( 'NONE',  ( 35.68042508330538709, -287.3584737447801558, -268.3145776192525318 ) ) ;
#27404=CARTESIAN_POINT ( 'NONE',  ( 17.05590036306628221, -277.7788697772809883, -320.0952223965823578 ) ) ;
#27405=CARTESIAN_POINT ( 'NONE',  ( -110.5017418172639907, -294.3803226888189783, -285.2388935552942257 ) ) ;
#27406=CARTESIAN_POINT ( 'NONE',  ( -109.7754286480210624, -298.5109648063378813, -255.0905864607733236 ) ) ;
#27407=CARTESIAN_POINT ( 'NONE',  ( -81.06816903332166646, -276.4562322859036385, -329.3113208726173866 ) ) ;
#27408=ORIENTED_EDGE ( 'NONE', *, *, #45253, .T. ) ;
#27410=CARTESIAN_POINT ( 'NONE',  ( -104.5865021315797350, -295.7317590908977536, -307.9384961836782963 ) ) ;
#27411=CARTESIAN_POINT ( 'NONE',  ( 35.94357302915922503, -289.6412678093057025, -283.4218583100583260 ) ) ;
#27413=CARTESIAN_POINT ( 'NONE',  ( 33.80220212180334016, -288.4249677313915754, -287.1670050828029161 ) ) ;
#27415=CARTESIAN_POINT ( 'NONE',  ( 3.706313439029678580, -279.6484947560007868, -205.4301429641734842 ) ) ;
#27416=CARTESIAN_POINT ( 'NONE',  ( -112.7902900871879126, -297.3905032902615062, -255.4332481503423935 ) ) ;
#27417=CARTESIAN_POINT ( 'NONE',  ( -63.93273379948281843, -289.8487573486725069, -199.3606468122460740 ) ) ;
#27418=CARTESIAN_POINT ( 'NONE',  ( -96.49244601821297351, -296.2224108746394791, -319.6455300220125082 ) ) ;
#27419=CARTESIAN_POINT ( 'NONE',  ( 34.50321368042285286, -293.7123695142064435, -257.2380349024562065 ) ) ;
#27423=CARTESIAN_POINT ( 'NONE',  ( 2.831726135935097144, -290.0439901617301643, -335.2984042817187742 ) ) ;
#27424=CARTESIAN_POINT ( 'NONE',  ( -19.05039376806008633, -285.3376638359844719, -350.3538533559490702 ) ) ;
#27426=CARTESIAN_POINT ( 'NONE',  ( 32.29655335312978792, -281.3203502777394647, -303.1028937768278979 ) ) ;
#27427=CARTESIAN_POINT ( 'NONE',  ( -37.51993876966864860, -285.0545814136198715, -345.2069844629641580 ) ) ;
#27428=CARTESIAN_POINT ( 'NONE',  ( 38.76950216745545674, -286.0345140429583921, -263.0319716620259669 ) ) ;
#27429=CARTESIAN_POINT ( 'NONE',  ( -106.0223964171046873, -289.0112535863611356, -241.5168748522592637 ) ) ;
#27430=CARTESIAN_POINT ( 'NONE',  ( 36.73266420422341838, -277.2094972349934210, -254.3846594581450802 ) ) ;
#27432=CARTESIAN_POINT ( 'NONE',  ( -78.63200210439875093, -277.6252152258310275, -330.6232601250132461 ) ) ;
#27433=CARTESIAN_POINT ( 'NONE',  ( 4.988920407950307556, -279.9900585380363509, -210.7623660415267750 ) ) ;
#27434=CARTESIAN_POINT ( 'NONE',  ( 39.07366994782440628, -276.7133764994251806, -276.8560179275592645 ) ) ;
#27435=CARTESIAN_POINT ( 'NONE',  ( -68.49690627285440314, -278.4467592661184767, -200.3656544439373590 ) ) ;
#27436=CARTESIAN_POINT ( 'NONE',  ( -64.69487635908569700, -181.8657373906415273, -359.8890228527233148 ) ) ;
#27437=CARTESIAN_POINT ( 'NONE',  ( -85.66942062355305154, -274.3430498377096001, -210.7184181443548709 ) ) ;
#27438=CARTESIAN_POINT ( 'NONE',  ( -62.66699936075727351, -299.1541419330542340, -198.2692633043302521 ) ) ;
#27439=CARTESIAN_POINT ( 'NONE',  ( -106.6379572354042296, -292.6233781216987495, -303.7686719486574702 ) ) ;
#27440=CARTESIAN_POINT ( 'NONE',  ( 82.65368334098262437, -299.1786464277133177, -192.8837611238190277 ) ) ;
#27442=CARTESIAN_POINT ( 'NONE',  ( 35.43272459205206104, -288.7479241839253064, -279.1990577936966247 ) ) ;
#27443=CARTESIAN_POINT ( 'NONE',  ( 38.34317685933614683, -289.2194144009057482, -263.0324034710992009 ) ) ;
#27444=CARTESIAN_POINT ( 'NONE',  ( 35.09830811078096247, -286.7665630169072415, -260.1758885920074817 ) ) ;
#27445=CARTESIAN_POINT ( 'NONE',  ( -112.2983557409630606, -284.2769706189415047, -253.0109974377302535 ) ) ;
#27446=CARTESIAN_POINT ( 'NONE',  ( -72.49300536962913100, -277.9784877313607581, -205.4702391460896820 ) ) ;
#27447=CARTESIAN_POINT ( 'NONE',  ( 16.86041374672074156, -288.6947358634152465, -219.6176547815807112 ) ) ;
#27448=CARTESIAN_POINT ( 'NONE',  ( 3.100503244290429894, -279.0856411858003980, -208.6952022770793178 ) ) ;
#27449=CARTESIAN_POINT ( 'NONE',  ( -85.41525797936425590, -279.0479800624798941, -326.0178727197855437 ) ) ;
#27450=CARTESIAN_POINT ( 'NONE',  ( -11.22619375635359162, -277.1947582623361654, -338.5957775671961940 ) ) ;
#27451=CARTESIAN_POINT ( 'NONE',  ( -70.48125557083621118, -288.2742195928282740, -339.4391138334882498 ) ) ;
#27452=CARTESIAN_POINT ( 'NONE',  ( -85.99222072904312597, -284.5098016705559303, -329.8362023898341135 ) ) ;
#27453=CARTESIAN_POINT ( 'NONE',  ( -110.1644125489615789, -284.7314306668059203, -295.1881085137200103 ) ) ;
#27454=CARTESIAN_POINT ( 'NONE',  ( 34.48583090488907033, -281.8916569509727310, -283.4621278111322340 ) ) ;
#27457=CARTESIAN_POINT ( 'NONE',  ( 151.9709352735115147, -297.1570670221753971, -195.3611179825600175 ) ) ;
#27458=CARTESIAN_POINT ( 'NONE',  ( -113.1338198747053241, -292.4373615970634432, -268.4105386301732210 ) ) ;
#27459=CARTESIAN_POINT ( 'NONE',  ( -44.83198890635473077, -290.6441824661231976, -194.1692292640431106 ) ) ;
#27460=CARTESIAN_POINT ( 'NONE',  ( -87.48570583729120642, -272.3906995855119249, -216.9157923600974698 ) ) ;
#27461=CARTESIAN_POINT ( 'NONE',  ( 39.13477531981056501, -293.0075702591530558, -278.8918126578204237 ) ) ;
#27462=CARTESIAN_POINT ( 'NONE',  ( -34.57114541367115379, -287.4967241094559540, -344.0524085595006909 ) ) ;
#27463=CARTESIAN_POINT ( 'NONE',  ( -4.361680243343561081, -290.7327275512591882, -204.0877174320054337 ) ) ;
#27464=CARTESIAN_POINT ( 'NONE',  ( -29.11345369632673297, -290.1506324523894591, -343.2955163495398665 ) ) ;
#27466=CARTESIAN_POINT ( 'NONE',  ( -104.7056410641375663, -292.1162448231181088, -303.4502878716615442 ) ) ;
#27467=CARTESIAN_POINT ( 'NONE',  ( -110.8417835582008593, -288.7543947888402727, -254.5599007528447260 ) ) ;
#27468=CARTESIAN_POINT ( 'NONE',  ( -85.66443643068748770, -293.3840823987449653, -212.9363270392000231 ) ) ;
#27469=CARTESIAN_POINT ( 'NONE',  ( -68.88711278083134459, -286.5681490517861221, -204.2542014814545155 ) ) ;
#27470=CARTESIAN_POINT ( 'NONE',  ( 20.77518091916995147, -294.8965061037041551, -222.6908277792020954 ) ) ;
#27473=CARTESIAN_POINT ( 'NONE',  ( -8.347270493903321764, -276.4096228299575841, -200.7519482697563262 ) ) ;
#27475=CARTESIAN_POINT ( 'NONE',  ( -112.9783591683269748, -295.9189796037368296, -256.8239605997793547 ) ) ;
#27476=CARTESIAN_POINT ( 'NONE',  ( 16.19506163846669367, -273.0642784632775601, -219.1812377889535526 ) ) ;
#27477=CARTESIAN_POINT ( 'NONE',  ( -111.6068375098344916, -276.5568804823640221, -276.1673229430492142 ) ) ;
#27478=CARTESIAN_POINT ( 'NONE',  ( -67.23319308046851006, -274.8563432785620080, -203.3128119753083354 ) ) ;
#27479=CARTESIAN_POINT ( 'NONE',  ( -7.900697975683619312, -273.0050082660452517, -199.7937159872668360 ) ) ;
#27480=CARTESIAN_POINT ( 'NONE',  ( -97.65599281484479377, -297.3942267175535790, -312.5222495544011281 ) ) ;
#27482=CARTESIAN_POINT ( 'NONE',  ( -101.3607911697761068, -297.8379242799479698, -234.9470288552004149 ) ) ;
#27484=CARTESIAN_POINT ( 'NONE',  ( 13.16359611347443348, -284.7735701835686086, -214.3659444510310266 ) ) ;
#27485=CARTESIAN_POINT ( 'NONE',  ( -110.3417001280813707, -272.3854989502048056, -270.3590007205843904 ) ) ;
#27486=CARTESIAN_POINT ( 'NONE',  ( -85.15486556093594572, -289.3582838214090884, -330.7586053970208582 ) ) ;
#27487=CARTESIAN_POINT ( 'NONE',  ( -97.78847990832565529, -299.1437673785420088, -225.3440886167354904 ) ) ;
#27488=CARTESIAN_POINT ( 'NONE',  ( 34.08938311030586732, -291.8403679688487955, -292.6687125254013608 ) ) ;
#27489=CARTESIAN_POINT ( 'NONE',  ( 36.83182285110126486, -280.4970021625206869, -250.2501067776279911 ) ) ;
#27490=CARTESIAN_POINT ( 'NONE',  ( 10.59707575819633618, -285.9094976428776249, -330.5268031993606428 ) ) ;
#27492=CARTESIAN_POINT ( 'NONE',  ( 6.067174800044488947, -287.2435990869718125, -329.6089059913525716 ) ) ;
#27494=CARTESIAN_POINT ( 'NONE',  ( -83.80469963662763178, -287.6899482727729946, -329.2354784656934044 ) ) ;
#27495=CARTESIAN_POINT ( 'NONE',  ( -111.0350334602965603, -274.0720295093142909, -270.3804279068866663 ) ) ;
#27496=CARTESIAN_POINT ( 'NONE',  ( 21.50522250096071986, -282.3171204041229885, -221.6205189710047705 ) ) ;
#27497=CARTESIAN_POINT ( 'NONE',  ( -110.0286478122418146, -294.8288559109639095, -250.2935782761344115 ) ) ;
#27498=CARTESIAN_POINT ( 'NONE',  ( 11.91668871776623639, -282.3443829044886684, -324.2370043169051996 ) ) ;
#27499=CARTESIAN_POINT ( 'NONE',  ( -111.6226369167017367, -296.9750813353718399, -249.8824974785207473 ) ) ;
#27500=CARTESIAN_POINT ( 'NONE',  ( -73.20103158731048154, -299.0875970637274577, -205.9808717845649255 ) ) ;
#27501=CARTESIAN_POINT ( 'NONE',  ( 5.032736954301892496, -282.6251541127557516, -208.4789094859022498 ) ) ;
#27502=CARTESIAN_POINT ( 'NONE',  ( -49.98278955158966852, -296.9456245938511074, -198.2250569196252741 ) ) ;
#27508=CARTESIAN_POINT ( 'NONE',  ( -92.87216662424697233, -285.8336180713416184, -320.2623451598472570 ) ) ;
#27510=CARTESIAN_POINT ( 'NONE',  ( -106.6379572354042296, -288.4809262143061801, -236.9535640164627353 ) ) ;
#27511=CARTESIAN_POINT ( 'NONE',  ( 36.33571411541639407, -275.0240808073210701, -292.2203004953053096 ) ) ;
#27514=CARTESIAN_POINT ( 'NONE',  ( -30.80485956688695026, -291.9704018938274999, -197.6543801931254905 ) ) ;
#27516=CARTESIAN_POINT ( 'NONE',  ( 34.62162197104575512, -283.2797118954034090, -286.2352487337064986 ) ) ;
#27517=CARTESIAN_POINT ( 'NONE',  ( 33.62370734642519920, -276.8851948664911333, -249.9215662272306417 ) ) ;
#27518=CARTESIAN_POINT ( 'NONE',  ( -94.87899353602283270, -285.2921221856511238, -320.6409962755051879 ) ) ;
#27520=CARTESIAN_POINT ( 'NONE',  ( -4.664089697125836764, -281.4066399955497673, -336.0825321686388634 ) ) ;
#27521=CARTESIAN_POINT ( 'NONE',  ( -110.1064407785872277, -280.3182582730640320, -288.5879567357413293 ) ) ;
#27522=CARTESIAN_POINT ( 'NONE',  ( -18.55202796198441817, -274.4542557106599361, -195.6338162350585606 ) ) ;
#27523=CARTESIAN_POINT ( 'NONE',  ( 35.73063161786891584, -275.0779566175285140, -245.9147612736157669 ) ) ;
#27524=CARTESIAN_POINT ( 'NONE',  ( -23.22219826375168594, -296.7904972994708146, -343.5024141261557702 ) ) ;
#27527=CARTESIAN_POINT ( 'NONE',  ( -104.1530215763134635, -295.1622821068463622, -234.5210099813571105 ) ) ;
#27528=CARTESIAN_POINT ( 'NONE',  ( 31.31744144402193797, -275.3940920659171638, -295.4863031157839828 ) ) ;
#27529=CARTESIAN_POINT ( 'NONE',  ( 39.01779417808786832, -295.0713897097376162, -270.2910974489604996 ) ) ;
#27530=CARTESIAN_POINT ( 'NONE',  ( 1.580966553772762406, -295.7489465650217539, -336.3386500434745585 ) ) ;
#27531=CARTESIAN_POINT ( 'NONE',  ( -85.01611820745596049, -293.3926104220229263, -212.6794199822438429 ) ) ;
#27532=CARTESIAN_POINT ( 'NONE',  ( -95.03534499213677122, -275.8927509631027419, -318.0411640013697934 ) ) ;
#27533=CARTESIAN_POINT ( 'NONE',  ( -110.7010874838116194, -280.3078465204497434, -283.0741390038166401 ) ) ;
#27534=CARTESIAN_POINT ( 'NONE',  ( -91.47082283380068191, -293.9095507372211387, -321.5367718840875568 ) ) ;
#27535=CARTESIAN_POINT ( 'NONE',  ( 36.66420507357636183, -283.6196196522857349, -286.6516883121927322 ) ) ;
#27536=CARTESIAN_POINT ( 'NONE',  ( -38.61655091987873334, -284.9561557716685911, -197.0505558027613802 ) ) ;
#27537=CARTESIAN_POINT ( 'NONE',  ( -111.2915329965731814, -274.0799573519071828, -284.0611421460235420 ) ) ;
#27539=CARTESIAN_POINT ( 'NONE',  ( -109.8942584414632506, -284.1041937039935306, -279.0566610771871865 ) ) ;
#27541=CARTESIAN_POINT ( 'NONE',  ( 23.16754149100059479, -283.2640251823428343, -317.5005377996771472 ) ) ;
#27542=CARTESIAN_POINT ( 'NONE',  ( -113.9436227052690072, -283.3520140231308915, -269.9684668169209658 ) ) ;
#27544=CARTESIAN_POINT ( 'NONE',  ( -113.0650911497885005, -279.3353231721430348, -282.9622395735897840 ) ) ;
#27545=CARTESIAN_POINT ( 'NONE',  ( -113.3863934105324063, -279.9848603097133264, -277.2875802944731731 ) ) ;
#27546=CARTESIAN_POINT ( 'NONE',  ( 8.479139178526475362, -281.3123447839362257, -208.5392560358893945 ) ) ;
#27547=CARTESIAN_POINT ( 'NONE',  ( 90.32002540683689062, -302.2645883696979467, -200.3030568020284647 ) ) ;
#27548=CARTESIAN_POINT ( 'NONE',  ( -109.1987091961355105, -267.5305874205028545, -307.0464688485295142 ) ) ;
#27550=CARTESIAN_POINT ( 'NONE',  ( -13.50499136230118857, -276.3625292218551408, -199.4256561863484478 ) ) ;
#27551=CARTESIAN_POINT ( 'NONE',  ( -71.60599505142221233, -195.9056560659656157, -360.2227879542884921 ) ) ;
#27552=CARTESIAN_POINT ( 'NONE',  ( -96.90943078455200066, -277.1905090651634396, -225.3562214412502840 ) ) ;
#27553=CARTESIAN_POINT ( 'NONE',  ( 27.17991173863390486, -294.7790864171419685, -230.1252792525458233 ) ) ;
#27554=CARTESIAN_POINT ( 'NONE',  ( 35.80994277582180274, -292.9061046636203400, -270.7687586548724425 ) ) ;
#27555=CARTESIAN_POINT ( 'NONE',  ( -112.8633468051969970, -290.2446218697569407, -255.5953112637739935 ) ) ;
#27557=CARTESIAN_POINT ( 'NONE',  ( -19.44305090082077925, -293.4011539718557060, -344.7004690562007454 ) ) ;
#27558=CARTESIAN_POINT ( 'NONE',  ( -4.217421090718192822, -284.8962691664578983, -204.4124822453422325 ) ) ;
#27559=CARTESIAN_POINT ( 'NONE',  ( -77.95032455262003168, -293.3604789860931419, -208.2176943468571437 ) ) ;
#27560=CARTESIAN_POINT ( 'NONE',  ( -97.77091240416136486, -286.4464078370949096, -228.5111983569666734 ) ) ;
#27562=CARTESIAN_POINT ( 'NONE',  ( -27.88998671274746854, -293.1104793945594906, -194.1269984574122134 ) ) ;
#27563=CARTESIAN_POINT ( 'NONE',  ( -66.57844489734239346, -283.9380611388800162, -337.3314111948610048 ) ) ;
#27564=CARTESIAN_POINT ( 'NONE',  ( 1.554527671027237989, -293.3391839350978785, -336.3542402111345382 ) ) ;
#27565=CARTESIAN_POINT ( 'NONE',  ( 16.57994092810535491, -289.1121046293197310, -325.1764671271653810 ) ) ;
#27566=CARTESIAN_POINT ( 'NONE',  ( -102.2459730535420874, -290.5013852880882723, -311.7745466030323769 ) ) ;
#27567=CARTESIAN_POINT ( 'NONE',  ( 10.11687371408157432, -288.5432702663702003, -325.8958201078382899 ) ) ;
#27570=CARTESIAN_POINT ( 'NONE',  ( -109.6416740960722080, -298.7037897777284456, -247.5371003688834151 ) ) ;
#27571=CARTESIAN_POINT ( 'NONE',  ( -37.23733949140996202, -296.7382676063367057, -193.8535291003551890 ) ) ;
#27572=CARTESIAN_POINT ( 'NONE',  ( -3.028269771781935127, -279.5759642878047657, -205.6476126200663259 ) ) ;
#27573=CARTESIAN_POINT ( 'NONE',  ( -71.36993810734335852, -273.1224594234291203, -201.3567273717213197 ) ) ;
#27574=CARTESIAN_POINT ( 'NONE',  ( -39.73072626825614151, -293.5625392248066419, -344.0282676493075087 ) ) ;
#27575=CARTESIAN_POINT ( 'NONE',  ( 24.62988793403597043, -276.7592097233517734, -229.8951287291834831 ) ) ;
#27576=CARTESIAN_POINT ( 'NONE',  ( -81.79198737790059681, -271.5794588559407998, -210.8404500025061452 ) ) ;
#27578=CARTESIAN_POINT ( 'NONE',  ( -73.48464267762841473, -296.7482661672439690, -334.2424001322260665 ) ) ;
#27579=CARTESIAN_POINT ( 'NONE',  ( -23.44682825410629690, -295.9501498990190385, -342.3932076799439983 ) ) ;
#27581=CARTESIAN_POINT ( 'NONE',  ( -63.96736559493859886, -296.9938349776746804, -341.7579971404136359 ) ) ;
#27583=CARTESIAN_POINT ( 'NONE',  ( -100.0068637073478186, -295.1116386563899709, -228.8273835354135315 ) ) ;
#27584=CARTESIAN_POINT ( 'NONE',  ( 12.96730746947797108, -293.4289607138384213, -217.3243720177621014 ) ) ;
#27585=CARTESIAN_POINT ( 'NONE',  ( -29.86478826530026609, -274.9473554526223325, -193.8872361055482543 ) ) ;
#27586=CARTESIAN_POINT ( 'NONE',  ( -75.26784763849518356, -290.1110113719590231, -207.2383149908752102 ) ) ;
#27587=CARTESIAN_POINT ( 'NONE',  ( -51.97598062056112411, -275.8651589376317474, -196.7495040150124055 ) ) ;
#27588=CARTESIAN_POINT ( 'NONE',  ( -85.77435706258641801, -273.8942172896033753, -210.5798111607869885 ) ) ;
#27590=CARTESIAN_POINT ( 'NONE',  ( -95.61864146156943889, -296.2672931152511069, -314.3804144753287346 ) ) ;
#27592=CARTESIAN_POINT ( 'NONE',  ( -8.196931093351738085, -282.4117920468839884, -200.8561935027971970 ) ) ;
#27593=CARTESIAN_POINT ( 'NONE',  ( 38.30968493627192828, -280.0890452723554063, -258.6079853689292918 ) ) ;
#27594=CARTESIAN_POINT ( 'NONE',  ( -99.57216309763640538, -277.3003594425779283, -315.5574229866656992 ) ) ;
#27595=CARTESIAN_POINT ( 'NONE',  ( 36.41230483756002911, -280.1942506987561501, -289.5128063912928837 ) ) ;
#27596=CARTESIAN_POINT ( 'NONE',  ( -1.277964097544683986, -280.5748210313462323, -336.3259483538149652 ) ) ;
#27597=CARTESIAN_POINT ( 'NONE',  ( 22.77257207110082149, -273.5389236089415590, -227.8934591347680225 ) ) ;
#27598=CARTESIAN_POINT ( 'NONE',  ( -81.68449435463507768, -279.6555729793868750, -330.9119404235894990 ) ) ;
#27601=CARTESIAN_POINT ( 'NONE',  ( -94.79007543861693819, -295.4735565898628238, -220.5467333199635505 ) ) ;
#27602=CARTESIAN_POINT ( 'NONE',  ( 10.10318621292782204, -290.7221492208485643, -211.7500544161656535 ) ) ;
#27603=CARTESIAN_POINT ( 'NONE',  ( -19.38677432578216653, -292.2768278923069829, -195.4289250637597206 ) ) ;
#27604=CARTESIAN_POINT ( 'NONE',  ( -34.33823053107608558, -279.0146256596172520, -345.4677594956069697 ) ) ;
#27605=CARTESIAN_POINT ( 'NONE',  ( -36.69389282156906518, -272.0601337845139369, -195.3511557099496372 ) ) ;
#27607=CARTESIAN_POINT ( 'NONE',  ( -44.26250081192613806, -285.0590500688032876, -345.6558632286009924 ) ) ;
#27609=CARTESIAN_POINT ( 'NONE',  ( -80.22184159682915094, -283.4717775772102186, -208.7656702330205860 ) ) ;
#27611=CARTESIAN_POINT ( 'NONE',  ( -47.86505605325606894, -293.9837412655173239, -343.0514383758520580 ) ) ;
#27612=CARTESIAN_POINT ( 'NONE',  ( 36.50552166033610746, -285.5934042910004109, -262.7813216009982966 ) ) ;
#27614=CARTESIAN_POINT ( 'NONE',  ( -71.87372008138898138, -293.5084023882123461, -336.9528128238608815 ) ) ;
#27615=CARTESIAN_POINT ( 'NONE',  ( -113.2165305978939358, -282.9297264235336797, -278.4677728390816469 ) ) ;
#27616=CARTESIAN_POINT ( 'NONE',  ( -93.71433507312700328, -280.8219783564400700, -222.7122017083493688 ) ) ;
#27617=CARTESIAN_POINT ( 'NONE',  ( -60.40506835693592791, -286.9647725944641365, -197.2572805548575730 ) ) ;
#27618=CARTESIAN_POINT ( 'NONE',  ( 38.17831918871550556, -279.6795977643929518, -261.4908110275704303 ) ) ;
#27619=CARTESIAN_POINT ( 'NONE',  ( 15.02949583536310918, -286.8168700710117491, -219.5058544068149615 ) ) ;
#27620=CARTESIAN_POINT ( 'NONE',  ( -110.9814983762989442, -279.9735419037218094, -270.6584032288535013 ) ) ;
#27621=CARTESIAN_POINT ( 'NONE',  ( -106.4132771030820663, -279.0330385724807343, -294.6335500764914741 ) ) ;
#27623=CARTESIAN_POINT ( 'NONE',  ( -37.99405631378817105, -288.0239039503819072, -195.0087375376406555 ) ) ;
#27625=CARTESIAN_POINT ( 'NONE',  ( -73.27873688191642998, -297.4226936028829869, -202.2028651255565421 ) ) ;
#27626=CARTESIAN_POINT ( 'NONE',  ( -109.7091805230882642, -292.7688189929253895, -252.0116696546971866 ) ) ;
#27628=CARTESIAN_POINT ( 'NONE',  ( -55.56934967048406548, -291.7662352645559167, -350.3683826091709648 ) ) ;
#27629=ORIENTED_EDGE ( 'NONE', *, *, #87430, .F. ) ;
#27630=CARTESIAN_POINT ( 'NONE',  ( -13.61642214219629388, -272.3592773142192982, -199.0369312755754265 ) ) ;
#27632=CARTESIAN_POINT ( 'NONE',  ( -19.49463162005092087, -293.2263260178216910, -344.4959440713471963 ) ) ;
#27633=CARTESIAN_POINT ( 'NONE',  ( -65.59072381180652656, -297.1801351323019276, -202.9817361014126789 ) ) ;
#27634=CARTESIAN_POINT ( 'NONE',  ( -53.54228963306366040, -290.7839182215230949, -342.2516503924534277 ) ) ;
#27635=CARTESIAN_POINT ( 'NONE',  ( -11.40880824863868526, -282.1546804486543465, -200.9855071766168919 ) ) ;
#27636=CARTESIAN_POINT ( 'NONE',  ( -74.12759924740237238, -290.9563645807033367, -337.3492128304811217 ) ) ;
#27637=CARTESIAN_POINT ( 'NONE',  ( -112.6892721554205394, -292.0343267173346362, -257.0930486787603400 ) ) ;
#27638=CARTESIAN_POINT ( 'NONE',  ( -40.07153979562591672, -288.0179972238098003, -195.4108102660858606 ) ) ;
#27639=CARTESIAN_POINT ( 'NONE',  ( -62.04963915970403576, -279.9063971833180062, -197.3767164906247444 ) ) ;
#27640=CARTESIAN_POINT ( 'NONE',  ( -30.74155502696780928, -293.0491720647729039, -345.6323095663776144 ) ) ;
#27641=CARTESIAN_POINT ( 'NONE',  ( 38.66750327269723186, -281.5404891994229502, -282.7561024184780081 ) ) ;
#27642=CARTESIAN_POINT ( 'NONE',  ( 26.44888698417057782, -277.9258663280769497, -308.3298745400100529 ) ) ;
#27643=CARTESIAN_POINT ( 'NONE',  ( -69.85430415644619018, -297.9805209788416391, -337.9475929042657754 ) ) ;
#27644=CARTESIAN_POINT ( 'NONE',  ( 37.49803502612482475, -273.6243876975385660, -257.1341533668179977 ) ) ;
#27647=CARTESIAN_POINT ( 'NONE',  ( 13.38233414402698251, -280.2926585656831548, -217.7067638255011843 ) ) ;
#27649=CARTESIAN_POINT ( 'NONE',  ( -37.11266466071617742, -278.2543790046399863, -346.9766961103813401 ) ) ;
#27650=CARTESIAN_POINT ( 'NONE',  ( -16.51685545203067207, -275.6419905724877708, -199.8270722053946997 ) ) ;
#27651=CARTESIAN_POINT ( 'NONE',  ( -97.38883146410131531, -284.2531725154895526, -222.5368330158063088 ) ) ;
#27652=CARTESIAN_POINT ( 'NONE',  ( -86.62019348327432056, -293.1167054582231231, -215.0688958986046373 ) ) ;
#27653=CARTESIAN_POINT ( 'NONE',  ( -108.4277388919072109, -274.5052111951486609, -242.7710011707785327 ) ) ;
#27655=CARTESIAN_POINT ( 'NONE',  ( -31.31571669936070279, -275.4418987109212935, -194.0787549732181390 ) ) ;
#27657=CARTESIAN_POINT ( 'NONE',  ( 32.51577207138818437, -275.6665440664735343, -291.5924990400104093 ) ) ;
#27658=CARTESIAN_POINT ( 'NONE',  ( -102.8309847285540855, -299.0350594090631375, -234.1508704494058009 ) ) ;
#27659=CARTESIAN_POINT ( 'NONE',  ( -74.73442363393843380, -281.5504951717720132, -335.2415685310998583 ) ) ;
#27661=CARTESIAN_POINT ( 'NONE',  ( -97.44439548734553114, -290.8633287890763199, -222.2631938877581206 ) ) ;
#27662=CARTESIAN_POINT ( 'NONE',  ( 36.32636387201440442, -273.7315544114858312, -282.7087091169038331 ) ) ;
#27663=CARTESIAN_POINT ( 'NONE',  ( 18.07712842093451400, -289.8739412439222178, -322.6601988303125950 ) ) ;
#27664=CARTESIAN_POINT ( 'NONE',  ( -88.13489411781456795, -290.2414784701313124, -217.4300511501999154 ) ) ;
#27666=CARTESIAN_POINT ( 'NONE',  ( -113.2305918655839747, -289.0090099640698895, -279.7139975508565612 ) ) ;
#27667=CARTESIAN_POINT ( 'NONE',  ( -109.8110189791233324, -290.1007034199903956, -279.3213251243636819 ) ) ;
#27669=CARTESIAN_POINT ( 'NONE',  ( 4.997521423533825669, -287.6892176130587018, -206.3534999519835651 ) ) ;
#27670=CARTESIAN_POINT ( 'NONE',  ( -100.8322833111559049, -279.3792902346340838, -234.2912783131542085 ) ) ;
#27671=CARTESIAN_POINT ( 'NONE',  ( -44.77938748352222120, -294.0643969775455275, -346.7436845850107829 ) ) ;
#27672=CARTESIAN_POINT ( 'NONE',  ( -111.7742044345890378, -284.9608910494137604, -289.7294870724063571 ) ) ;
#27673=CARTESIAN_POINT ( 'NONE',  ( -85.50298577752880647, -285.7399204422563344, -210.3091833257372514 ) ) ;
#27674=CARTESIAN_POINT ( 'NONE',  ( 24.15053851264908147, -282.4311609880903688, -309.8341772453737804 ) ) ;
#27675=CARTESIAN_POINT ( 'NONE',  ( 84.52794612516449035, 83.35382402778485300, -302.3197191937509842 ) ) ;
#27676=CARTESIAN_POINT ( 'NONE',  ( -96.29398733087926132, -239.0646663885169971, -340.8987983896206515 ) ) ;
#27677=CARTESIAN_POINT ( 'NONE',  ( -56.32650456138331663, -169.0553163394745297, -360.7103527500878499 ) ) ;
#27678=CARTESIAN_POINT ( 'NONE',  ( 24.11448446657037081, -275.2987689420457400, -310.1500906038724565 ) ) ;
#27679=CARTESIAN_POINT ( 'NONE',  ( -0.3785840698713352492, -273.4763231492167392, -207.0380590452716945 ) ) ;
#27680=CARTESIAN_POINT ( 'NONE',  ( 8.864193877305035940, -293.9448730891281230, -331.8797514379827476 ) ) ;
#27681=CARTESIAN_POINT ( 'NONE',  ( -54.38370458779698424, -170.1712701406207486, -361.1722839838796517 ) ) ;
#27682=CARTESIAN_POINT ( 'NONE',  ( 22.38394935977466105, -273.5921984346008458, -222.5266875958565720 ) ) ;
#27683=CARTESIAN_POINT ( 'NONE',  ( -44.71495253834831374, -299.8184124375551391, -196.4417532559928077 ) ) ;
#27684=CARTESIAN_POINT ( 'NONE',  ( -33.50595437956121714, -293.1812074276649014, -197.1398770807768983 ) ) ;
#27686=CARTESIAN_POINT ( 'NONE',  ( -114.1027984822798089, -297.5027397814274650, -269.6168117708892282 ) ) ;
#27687=CARTESIAN_POINT ( 'NONE',  ( 35.69179780106460242, -288.0892547718623860, -273.7564419364115906 ) ) ;
#27689=CARTESIAN_POINT ( 'NONE',  ( 36.12957975802836330, -294.0718971154751102, -247.8637880870911374 ) ) ;
#27690=CARTESIAN_POINT ( 'NONE',  ( -92.64840805114447164, -296.3111780202609111, -323.8465829417602322 ) ) ;
#27691=CARTESIAN_POINT ( 'NONE',  ( 12.90161958726231184, -292.9443056210603231, -217.4025603315702995 ) ) ;
#27693=CARTESIAN_POINT ( 'NONE',  ( 22.47755597598199984, -276.8442076921319881, -224.1776267369401410 ) ) ;
#27695=CARTESIAN_POINT ( 'NONE',  ( -110.4892203164836957, -278.3620329675359244, -246.3390350988140085 ) ) ;
#27696=CARTESIAN_POINT ( 'NONE',  ( -6.440566982790778106, -275.4095560453952203, -203.9643679174246529 ) ) ;
#27697=CARTESIAN_POINT ( 'NONE',  ( -3.035364976444239637, -276.2592069854427450, -202.5450663414689529 ) ) ;
#27698=CARTESIAN_POINT ( 'NONE',  ( -108.1989566239285665, -276.2395449046551903, -296.1587096935703585 ) ) ;
#27699=CARTESIAN_POINT ( 'NONE',  ( -65.61979572447937414, -298.3237107666147381, -202.9501249783413641 ) ) ;
#27700=CARTESIAN_POINT ( 'NONE',  ( -108.3999240650138773, -295.3781541007084002, -251.1787687992029134 ) ) ;
#27702=CARTESIAN_POINT ( 'NONE',  ( -113.2374326532378319, -278.8864908656411217, -282.9850907236757962 ) ) ;
#27703=CARTESIAN_POINT ( 'NONE',  ( -35.11550923842111160, -277.1901022697819030, -343.3271654200470948 ) ) ;
#27705=CARTESIAN_POINT ( 'NONE',  ( -37.96153848987580659, -284.7293711236492300, -193.8567777440656528 ) ) ;
#27706=CARTESIAN_POINT ( 'NONE',  ( -59.62938112530403600, -299.7644559211680644, -198.5205078157930814 ) ) ;
#27709=CARTESIAN_POINT ( 'NONE',  ( 29.56860480009935799, -287.1481684185879999, -300.0775266694301422 ) ) ;
#27710=CARTESIAN_POINT ( 'NONE',  ( 0.9430474256644593156, -278.8099815993402899, -206.9594410590462417 ) ) ;
#27711=CARTESIAN_POINT ( 'NONE',  ( -89.88165379784589959, -277.8674667091413539, -218.7629258732470419 ) ) ;
#27712=CARTESIAN_POINT ( 'NONE',  ( -68.40717075724357699, -281.5433517477497389, -338.0091093476349329 ) ) ;
#27713=CARTESIAN_POINT ( 'NONE',  ( -77.95547014114582396, -287.5069994248777334, -207.2488651788966081 ) ) ;
#27714=CARTESIAN_POINT ( 'NONE',  ( -7.331332943831510462, -277.8546272854011363, -337.3425211279961218 ) ) ;
#27717=CARTESIAN_POINT ( 'NONE',  ( -51.15075254707824115, -275.4661958800792263, -345.0824943266380274 ) ) ;
#27719=CARTESIAN_POINT ( 'NONE',  ( 35.70423805345799195, -276.2555875449469340, -274.3098780883924519 ) ) ;
#27720=CARTESIAN_POINT ( 'NONE',  ( 28.17669662114862206, -284.0431787711817719, -307.3097380317208831 ) ) ;
#27722=CARTESIAN_POINT ( 'NONE',  ( -3.679862741015699434, -290.5316854709591325, -338.0230535551716571 ) ) ;
#27725=CARTESIAN_POINT ( 'NONE',  ( -91.42594102420888191, -293.8212159059965529, -322.3954285541440186 ) ) ;
#27727=CARTESIAN_POINT ( 'NONE',  ( -5.076536440178148091, -273.1708663601064586, -204.3153676671505821 ) ) ;
#27728=CARTESIAN_POINT ( 'NONE',  ( 35.70275299060480023, -291.5190268903338620, -257.0474503475281836 ) ) ;
#27729=CARTESIAN_POINT ( 'NONE',  ( 64.33209501061345748, 48.33985520751024723, -319.1928417150128325 ) ) ;
#27731=CARTESIAN_POINT ( 'NONE',  ( -38.92536795428206631, -287.5515671899481731, -346.6513516374243409 ) ) ;
#27732=CARTESIAN_POINT ( 'NONE',  ( 37.97390402269154919, -285.6643135538512865, -260.2847205746248278 ) ) ;
#27734=CARTESIAN_POINT ( 'NONE',  ( -110.1981253010328317, -286.1129925509735017, -260.0017633558638295 ) ) ;
#27735=CARTESIAN_POINT ( 'NONE',  ( -52.13154334789275168, -286.6607744384797911, -198.7101426649522011 ) ) ;
#27737=CARTESIAN_POINT ( 'NONE',  ( -112.1769488774193064, -292.4136254876100338, -279.6275797635290132 ) ) ;
#27738=CARTESIAN_POINT ( 'NONE',  ( 21.50385362800916766, -274.2795883042095397, -317.7789904473227693 ) ) ;
#27739=CARTESIAN_POINT ( 'NONE',  ( 8.231962502020227390, -276.7812389605397811, -332.4656978067777118 ) ) ;
#27740=CARTESIAN_POINT ( 'NONE',  ( -85.57467267313248271, -289.4712467822806161, -212.1305440981531092 ) ) ;
#27741=CARTESIAN_POINT ( 'NONE',  ( -103.6057918900136201, -278.0400668303644238, -309.6839154718165332 ) ) ;
#27742=CARTESIAN_POINT ( 'NONE',  ( -111.6909798513124485, -298.6248778251186877, -263.1656264632775333 ) ) ;
#27745=CARTESIAN_POINT ( 'NONE',  ( -80.93201050390715068, -282.3424669813427386, -329.5947774082359274 ) ) ;
#27746=CARTESIAN_POINT ( 'NONE',  ( -71.57071146206192225, -277.5998769881154544, -203.6132336864991430 ) ) ;
#27748=CARTESIAN_POINT ( 'NONE',  ( 19.53216446816905716, -273.3351467189945083, -219.4103534795385144 ) ) ;
#27749=CARTESIAN_POINT ( 'NONE',  ( -108.2730038300416595, -277.6671135310381828, -288.0944539993737408 ) ) ;
#27750=CARTESIAN_POINT ( 'NONE',  ( 18.51045061406193426, -295.7506505319004759, -318.4557745035315861 ) ) ;
#27751=AXIS2_PLACEMENT_3D ( 'NONE', #66303, #9914, #89429 ) ;
#27752=CARTESIAN_POINT ( 'NONE',  ( 37.68514430102204926, -280.2721798262482480, -254.4090895892437345 ) ) ;
#27753=CARTESIAN_POINT ( 'NONE',  ( -68.60693562699356107, -296.4146222192179039, -336.6009713808896322 ) ) ;
#27754=CARTESIAN_POINT ( 'NONE',  ( -101.2073047603732903, -297.3087404217823746, -312.5815087232940073 ) ) ;
#27755=CARTESIAN_POINT ( 'NONE',  ( -103.2223275882264062, -272.6446705769380401, -238.8677788116357306 ) ) ;
#27756=CARTESIAN_POINT ( 'NONE',  ( -36.20056714911405038, -294.0665827818957609, -195.3569767363293010 ) ) ;
#27757=CARTESIAN_POINT ( 'NONE',  ( -112.9986466442123572, -284.9013320331508794, -255.7649088036768603 ) ) ;
#27758=CARTESIAN_POINT ( 'NONE',  ( 1.800476435031018951, -272.7094804265789776, -205.4905122053528714 ) ) ;
#27759=CARTESIAN_POINT ( 'NONE',  ( 38.67463123557805460, -287.5429613925635408, -282.9537771995813955 ) ) ;
#27760=CARTESIAN_POINT ( 'NONE',  ( -71.72116591213416825, -281.5754793454692617, -204.0903970262988310 ) ) ;
#27761=ADVANCED_FACE ( 'NONE', ( #12582 ), #85046, .T. ) ;
#27762=CARTESIAN_POINT ( 'NONE',  ( -77.16699619046305259, -284.5629841276941647, -208.8407701021576202 ) ) ;
#27763=CARTESIAN_POINT ( 'NONE',  ( -64.74075229874868853, -287.4096252036816281, -340.2321406871787417 ) ) ;
#27764=CARTESIAN_POINT ( 'NONE',  ( 69.94643833976951441, 44.42656045538938514, -317.4108715071801612 ) ) ;
#27765=CARTESIAN_POINT ( 'NONE',  ( -9.464111096576960591, -285.9342049204319665, -202.8136920183264351 ) ) ;
#27766=CARTESIAN_POINT ( 'NONE',  ( 17.66606512967681653, -283.2304255070220051, -323.9811409034066969 ) ) ;
#27768=CARTESIAN_POINT ( 'NONE',  ( -97.27233137253044504, -290.2554564205926795, -222.3909225182138130 ) ) ;
#27769=CARTESIAN_POINT ( 'NONE',  ( -97.08252839257366418, -280.7918564639961119, -223.0591745013976777 ) ) ;
#27770=CARTESIAN_POINT ( 'NONE',  ( -74.78131832722732497, -280.8796353169584563, -203.6410066050127909 ) ) ;
#27771=CARTESIAN_POINT ( 'NONE',  ( 34.48506770012869538, -281.5583507417507008, -283.4663118048673596 ) ) ;
#27772=CARTESIAN_POINT ( 'NONE',  ( -10.80579484633922327, -276.3981916850656830, -200.1568545849455063 ) ) ;
#27773=CARTESIAN_POINT ( 'NONE',  ( -8.388037073456116488, -294.6835563454133649, -341.7666387349515276 ) ) ;
#27774=CARTESIAN_POINT ( 'NONE',  ( -110.5568734288250425, -288.3838469392683237, -284.9656979898983309 ) ) ;
#27775=CARTESIAN_POINT ( 'NONE',  ( -100.1545839252071488, -295.9915693547708884, -232.4633854209693311 ) ) ;
#27778=CARTESIAN_POINT ( 'NONE',  ( -23.77961776314300479, -284.7976793969160099, -343.5552715542814894 ) ) ;
#27779=CARTESIAN_POINT ( 'NONE',  ( -108.3205719654971517, -295.9920168870833095, -287.5628310995685979 ) ) ;
#27781=CARTESIAN_POINT ( 'NONE',  ( 10.91357574335173375, -293.7812204986319671, -210.6864219412660191 ) ) ;
#27782=CARTESIAN_POINT ( 'NONE',  ( -70.25339703745979136, -284.1491536326142295, -335.6492517785920313 ) ) ;
#27783=CARTESIAN_POINT ( 'NONE',  ( -46.83996842348226153, -272.9930901258628637, -194.1862985738517864 ) ) ;
#27784=CARTESIAN_POINT ( 'NONE',  ( 0.6761292927307080980, -289.2108532868189172, -337.2640755107474320 ) ) ;
#27785=CARTESIAN_POINT ( 'NONE',  ( -85.33846531074344455, -281.8469817804627837, -328.9837758017661713 ) ) ;
#27786=CARTESIAN_POINT ( 'NONE',  ( -93.57444636036071017, -290.1676445437156531, -323.0081031047207034 ) ) ;
#27787=CARTESIAN_POINT ( 'NONE',  ( 17.84429787934677236, -288.5673809809975410, -318.2551638927276940 ) ) ;
#27791=CARTESIAN_POINT ( 'NONE',  ( 202.2091371056811795, 292.1033490241518393, -68.21892602122903781 ) ) ;
#27792=CARTESIAN_POINT ( 'NONE',  ( 35.78497577281001440, -284.8380690714490129, -253.7030783399848985 ) ) ;
#27794=CARTESIAN_POINT ( 'NONE',  ( -43.76452800803483001, -278.8895441777788733, -197.2834616080425008 ) ) ;
#27795=CARTESIAN_POINT ( 'NONE',  ( 39.60983844573426182, -275.1932189243736389, -268.3105076929415418 ) ) ;
#27796=CARTESIAN_POINT ( 'NONE',  ( -35.03626274600039636, -279.0232862442031774, -345.1589347151418679 ) ) ;
#27797=CARTESIAN_POINT ( 'NONE',  ( 186.3940997172195750, 260.5663691252829608, -151.7046075576564590 ) ) ;
#27798=CARTESIAN_POINT ( 'NONE',  ( 32.64061832101208438, -279.7326540102445733, -239.6840679964911374 ) ) ;
#27799=CARTESIAN_POINT ( 'NONE',  ( -98.90283554046479253, -281.9965521890634363, -312.6658560471549890 ) ) ;
#27801=CARTESIAN_POINT ( 'NONE',  ( -96.60287615452892851, -297.6662759078676572, -317.9431062379033506 ) ) ;
#27802=CARTESIAN_POINT ( 'NONE',  ( 35.70373570007519248, -294.0856817030418711, -273.4853544332152069 ) ) ;
#27804=CARTESIAN_POINT ( 'NONE',  ( -107.4671840212320149, -289.5269946965645431, -248.3264842510507435 ) ) ;
#27805=CARTESIAN_POINT ( 'NONE',  ( 24.39307639438615283, -275.5931224610558843, -224.5121250317246506 ) ) ;
#27806=CARTESIAN_POINT ( 'NONE',  ( -107.1965291664068474, -272.8348866151536072, -248.9911961818465045 ) ) ;
#27814=CARTESIAN_POINT ( 'NONE',  ( 5.090934676742263854, -281.7208644691550035, -210.5807066730290558 ) ) ;
#27815=CARTESIAN_POINT ( 'NONE',  ( -96.91658063507647114, -280.9518433919937479, -223.1932514803793310 ) ) ;
#27816=CARTESIAN_POINT ( 'NONE',  ( -108.8922226143005645, -283.8170366458926992, -254.6843170608131288 ) ) ;
#27817=CARTESIAN_POINT ( 'NONE',  ( 27.52688981155101189, -282.9272361707023151, -234.2649752909618428 ) ) ;
#27818=CARTESIAN_POINT ( 'NONE',  ( 29.77785774090250115, -274.4382455516015398, -300.7859877772241930 ) ) ;
#27821=CARTESIAN_POINT ( 'NONE',  ( -28.60921274861700070, -277.7470460517150741, -346.7552815917981661 ) ) ;
#27826=CARTESIAN_POINT ( 'NONE',  ( -104.3105844749664044, -286.0757111728668178, -305.0230546044978723 ) ) ;
#27828=CARTESIAN_POINT ( 'NONE',  ( 35.06901717529549245, -292.6117123840389809, -259.9069443353192241 ) ) ;
#27829=CARTESIAN_POINT ( 'NONE',  ( 39.53832300489872864, -286.8798796672231219, -268.6953360801878148 ) ) ;
#27830=CARTESIAN_POINT ( 'NONE',  ( -110.1864277931821334, -282.9633835506042487, -257.1895688095265768 ) ) ;
#27831=CARTESIAN_POINT ( 'NONE',  ( -71.43521868467900049, -284.1672966304868169, -205.1460360545227672 ) ) ;
#27832=CARTESIAN_POINT ( 'NONE',  ( 25.08112882513839637, -286.3343455412088474, -310.1274911929752420 ) ) ;
#27833=CARTESIAN_POINT ( 'NONE',  ( -34.81759642637386776, -284.2248543295481795, -343.7272818156513381 ) ) ;
#27834=CARTESIAN_POINT ( 'NONE',  ( 1.407088039515917544, -272.5697584191947271, -206.1463839728284029 ) ) ;
#27835=CARTESIAN_POINT ( 'NONE',  ( -68.15835018713890747, -284.0540769866300366, -200.6563305972389344 ) ) ;
#27836=CARTESIAN_POINT ( 'NONE',  ( -110.6448680717878261, -298.3486259242654342, -286.2244789886882472 ) ) ;
#27837=CARTESIAN_POINT ( 'NONE',  ( -4.272386506592572353, -284.4868507060746197, -202.8454595614456082 ) ) ;
#27838=CARTESIAN_POINT ( 'NONE',  ( -93.27764968013811142, -280.1632085063107525, -223.0705004749699469 ) ) ;
#27839=CARTESIAN_POINT ( 'NONE',  ( 31.20372759903785820, -289.9559266745055197, -301.2083668266398604 ) ) ;
#27842=CARTESIAN_POINT ( 'NONE',  ( 7.967528631920097304, -294.5856262091520534, -209.8277574451288672 ) ) ;
#27843=CARTESIAN_POINT ( 'NONE',  ( -68.90158566030386567, -275.4669149974804441, -338.4118106373981618 ) ) ;
#27844=CARTESIAN_POINT ( 'NONE',  ( -100.5535876938750022, -289.1712039249697455, -314.0465399323989573 ) ) ;
#27845=CARTESIAN_POINT ( 'NONE',  ( -3.993190426808736593, -293.0046814795990713, -336.2108003082978485 ) ) ;
#27846=CARTESIAN_POINT ( 'NONE',  ( -102.5860235892323828, -277.6952922186414980, -236.4211052408278420 ) ) ;
#27847=CARTESIAN_POINT ( 'NONE',  ( -71.00688282303227084, -295.7426845041317165, -204.1841361142431595 ) ) ;
#27848=CARTESIAN_POINT ( 'NONE',  ( -68.02222776825142603, -292.9558717238584791, -203.5644417726997801 ) ) ;
#27849=CARTESIAN_POINT ( 'NONE',  ( 10.64812456238589888, -284.9090924074130839, -330.4860931364851808 ) ) ;
#27850=CARTESIAN_POINT ( 'NONE',  ( -110.1441692646284025, -294.7416971531197305, -293.2633282135773811 ) ) ;
#27851=CARTESIAN_POINT ( 'NONE',  ( 21.00233050910374999, -289.7820505990085280, -315.5746672302768161 ) ) ;
#27852=CARTESIAN_POINT ( 'NONE',  ( -8.869833837920655384, -290.6594074170397448, -199.9102354879851191 ) ) ;
#27853=CARTESIAN_POINT ( 'NONE',  ( -93.90429155225014313, -292.6401192679890073, -223.2665189243566886 ) ) ;
#27855=CARTESIAN_POINT ( 'NONE',  ( -22.71832305514859129, -293.0469688396767651, -198.6759830561543652 ) ) ;
#27857=CARTESIAN_POINT ( 'NONE',  ( 121.3395553409046670, -299.5541904835127980, -198.1000099699160444 ) ) ;
#27858=CARTESIAN_POINT ( 'NONE',  ( -111.2537441628948045, -292.0111517702345054, -250.1862362095788512 ) ) ;
#27859=CARTESIAN_POINT ( 'NONE',  ( 35.40392965850670493, -279.3201327872214392, -250.6530238920276474 ) ) ;
#27860=CARTESIAN_POINT ( 'NONE',  ( -33.50843596152530068, -292.1017104308021999, -197.4493385235594189 ) ) ;
#27861=CARTESIAN_POINT ( 'NONE',  ( 21.97070697205877465, -280.8920786936284344, -221.2587925387763050 ) ) ;
#27862=CARTESIAN_POINT ( 'NONE',  ( 6.909384276224850296, -282.1350184663884306, -333.4150734688782336 ) ) ;
#27863=CARTESIAN_POINT ( 'NONE',  ( 34.18854243352146938, -285.2605713027791126, -247.7697927691642121 ) ) ;
#27864=CARTESIAN_POINT ( 'NONE',  ( 35.43702946269367970, -279.8823841023202590, -285.0578981763972024 ) ) ;
#27865=CARTESIAN_POINT ( 'NONE',  ( -82.06236911663238232, -283.4427157167420432, -210.0878805667496749 ) ) ;
#27866=CARTESIAN_POINT ( 'NONE',  ( 19.62410622756333467, -279.3373208916834756, -219.5713490923693598 ) ) ;
#27868=CARTESIAN_POINT ( 'NONE',  ( 29.86732314095164398, -285.9909378734185452, -233.3125708335854256 ) ) ;
#27869=CARTESIAN_POINT ( 'NONE',  ( -11.44260362485885807, -275.2010569009327128, -201.8829939542681871 ) ) ;
#27871=CARTESIAN_POINT ( 'NONE',  ( 36.50864150966231847, -295.1572839987191514, -270.7439568554125344 ) ) ;
#27872=CARTESIAN_POINT ( 'NONE',  ( -2.839963049624011138, -275.9243922329022212, -202.1685529839888886 ) ) ;
#27873=CARTESIAN_POINT ( 'NONE',  ( -45.91479224835151030, -276.8304283633519844, -342.9278917448578454 ) ) ;
#27874=CARTESIAN_POINT ( 'NONE',  ( -92.81355847828376682, -291.4505834663241330, -216.8823302304002709 ) ) ;
#27875=CARTESIAN_POINT ( 'NONE',  ( 24.73310678854785394, -280.2122656931841789, -313.4655595692692032 ) ) ;
#27877=CARTESIAN_POINT ( 'NONE',  ( -79.59264351942204030, -291.3319410763273822, -205.9245798495138615 ) ) ;
#27879=CARTESIAN_POINT ( 'NONE',  ( -89.97712714218947383, -290.3443895934769898, -219.4403926232700712 ) ) ;
#27880=CARTESIAN_POINT ( 'NONE',  ( -33.56179022501933673, -293.0044396263564295, -345.2785891142985406 ) ) ;
#27881=ORIENTED_EDGE ( 'NONE', *, *, #63185, .F. ) ;
#27884=CARTESIAN_POINT ( 'NONE',  ( 32.68986847843369503, -292.7823885402426640, -249.3644386981601997 ) ) ;
#27886=CARTESIAN_POINT ( 'NONE',  ( -107.3417001280813565, -270.0523547857346784, -270.3292895737509980 ) ) ;
#27887=CARTESIAN_POINT ( 'NONE',  ( -104.4032088572309078, -295.1238861540036282, -307.8271991359120534 ) ) ;
#27888=CARTESIAN_POINT ( 'NONE',  ( -106.5523595750212564, -285.4469594962887982, -302.9676033856445656 ) ) ;
#27889=CARTESIAN_POINT ( 'NONE',  ( 20.34195925106324054, -286.7553234639853486, -225.6219243692896441 ) ) ;
#27890=CARTESIAN_POINT ( 'NONE',  ( 34.17742584323769961, -276.8400064867641390, -252.5925396873911950 ) ) ;
#27891=CARTESIAN_POINT ( 'NONE',  ( -112.0192357161708401, -294.5940575145658613, -268.6710504015970287 ) ) ;
#27892=CARTESIAN_POINT ( 'NONE',  ( -111.3977033364850229, -298.2974729872357784, -271.5007827338120592 ) ) ;
#27894=CARTESIAN_POINT ( 'NONE',  ( 33.96868166395599786, -274.5757362630392322, -287.7910098152834735 ) ) ;
#27897=CARTESIAN_POINT ( 'NONE',  ( -81.86293117527280572, -295.3068547626938880, -333.2243483208449675 ) ) ;
#27898=CARTESIAN_POINT ( 'NONE',  ( 26.95187574008452813, -289.9784902834215359, -307.9817439055210002 ) ) ;
#27899=CARTESIAN_POINT ( 'NONE',  ( -46.71249304810552871, -295.9331539542798737, -195.8971521768887385 ) ) ;
#27901=CARTESIAN_POINT ( 'NONE',  ( -66.36187284109030315, -290.0937235665642788, -337.5100811796905305 ) ) ;
#27903=CARTESIAN_POINT ( 'NONE',  ( 12.84741377223365610, -279.7916940393914729, -212.2760677698064455 ) ) ;
#27904=CARTESIAN_POINT ( 'NONE',  ( -114.2361169130283685, -297.2129476498462282, -269.6118159258965647 ) ) ;
#27905=CARTESIAN_POINT ( 'NONE',  ( -111.1091296955568168, -288.9114099761761736, -253.0789936976636341 ) ) ;
#27906=CARTESIAN_POINT ( 'NONE',  ( -110.3243136509194926, -296.5770805311212825, -294.8413633830983258 ) ) ;
#27907=CARTESIAN_POINT ( 'NONE',  ( 8.858937544581662493, -293.0391543083448482, -213.7483122041708441 ) ) ;
#27911=CARTESIAN_POINT ( 'NONE',  ( 36.12221546286342999, -289.3337391289682614, -291.0430546115063635 ) ) ;
#27912=CARTESIAN_POINT ( 'NONE',  ( -117.3452863284742733, -275.1604526064901393, -261.3791111993605227 ) ) ;
#27914=CARTESIAN_POINT ( 'NONE',  ( 33.08292177469775908, -280.5063885318763823, -239.4793204938449662 ) ) ;
#27915=CARTESIAN_POINT ( 'NONE',  ( -83.91633429756087992, -285.6932732906661272, -329.0008965336969595 ) ) ;
#27916=CARTESIAN_POINT ( 'NONE',  ( -12.87507038858997532, -284.9387818915158732, -197.9733405531459027 ) ) ;
#27917=CARTESIAN_POINT ( 'NONE',  ( -76.64947980478116563, -287.6625334759774546, -333.5767224956252903 ) ) ;
#27918=CARTESIAN_POINT ( 'NONE',  ( 33.55740889120653492, -277.0690759643125602, -243.6474170215644222 ) ) ;
#27919=CARTESIAN_POINT ( 'NONE',  ( -106.2642072771267721, -278.2303353700393700, -294.5703570492445351 ) ) ;
#27920=CARTESIAN_POINT ( 'NONE',  ( -41.04806842016684243, -279.3528599735148532, -197.3532040111178674 ) ) ;
#27921=CARTESIAN_POINT ( 'NONE',  ( 38.18527739032933965, -276.4637415639192568, -256.9757010926957719 ) ) ;
#27922=CARTESIAN_POINT ( 'NONE',  ( -110.1673777833031238, -277.6494193630538234, -246.4351457014333562 ) ) ;
#27923=CARTESIAN_POINT ( 'NONE',  ( 137.0730373049989055, 179.9819603676357929, -239.3176569815323376 ) ) ;
#27924=CARTESIAN_POINT ( 'NONE',  ( -81.12604869336394131, -274.4147922157858375, -207.2431406866963073 ) ) ;
#27925=CARTESIAN_POINT ( 'NONE',  ( 52.70517975663122456, -300.5839879508616832, -193.9289803200042286 ) ) ;
#27926=CARTESIAN_POINT ( 'NONE',  ( -85.28047601435908120, -286.1948066931273615, -330.5268031993605859 ) ) ;
#27928=CARTESIAN_POINT ( 'NONE',  ( 24.50648177546417728, -289.1737003427390960, -309.7188169580091426 ) ) ;
#27929=CARTESIAN_POINT ( 'NONE',  ( -23.98633205694595105, -287.9804894034323297, -195.5038196974234381 ) ) ;
#27930=CARTESIAN_POINT ( 'NONE',  ( 20.43292247756048141, -287.5308739620652432, -315.1696133570176244 ) ) ;
#27931=CARTESIAN_POINT ( 'NONE',  ( -111.4339028052273619, -283.7997974221494815, -291.0944825380661882 ) ) ;
#27932=CARTESIAN_POINT ( 'NONE',  ( -2.756337512046009408, -278.9171943879674700, -205.1525110326900290 ) ) ;
#27933=CARTESIAN_POINT ( 'NONE',  ( 21.30210453034180418, -288.7820913678932584, -224.8444214997742279 ) ) ;
#27934=CARTESIAN_POINT ( 'NONE',  ( 28.76454254570944258, -280.4705849856101167, -303.0448296655491163 ) ) ;
#27935=CARTESIAN_POINT ( 'NONE',  ( -68.22954056533076539, -278.7817129990770013, -337.0621727666297716 ) ) ;
#27937=CARTESIAN_POINT ( 'NONE',  ( -6.508708559273599370, -274.9607239073000642, -204.1243074254262240 ) ) ;
#27938=CARTESIAN_POINT ( 'NONE',  ( 27.10240031239158398, -286.8942965839950148, -311.8710490412135528 ) ) ;
#27939=CARTESIAN_POINT ( 'NONE',  ( 21.49297940993257328, -283.0218273886974316, -319.7841824839669016 ) ) ;
#27940=CARTESIAN_POINT ( 'NONE',  ( -86.05855980369636882, -284.1993662563010616, -329.9110506979000661 ) ) ;
#27941=CARTESIAN_POINT ( 'NONE',  ( 21.81318416493202150, -282.3174695549828925, -313.1575103015319428 ) ) ;
#27942=ORIENTED_EDGE ( 'NONE', *, *, #54431, .T. ) ;
#27945=CARTESIAN_POINT ( 'NONE',  ( 29.28789883055610233, -289.8879691579193718, -306.5375349091719954 ) ) ;
#27946=CARTESIAN_POINT ( 'NONE',  ( -88.30841731686322760, -290.0403525207105986, -213.3024463314751813 ) ) ;
#27948=CARTESIAN_POINT ( 'NONE',  ( -43.48996544767952344, -273.0314699460711267, -197.3334855143597508 ) ) ;
#27949=CARTESIAN_POINT ( 'NONE',  ( 26.42257728213035506, -293.4678031081490417, -313.3428549522618596 ) ) ;
#27950=CARTESIAN_POINT ( 'NONE',  ( -94.65561665588371909, -288.3830240674366223, -316.6841438649119027 ) ) ;
#27951=CARTESIAN_POINT ( 'NONE',  ( 34.08886541240971724, -292.0451003689444178, -289.7908993455463360 ) ) ;
#27952=CARTESIAN_POINT ( 'NONE',  ( 29.79444020040299179, -289.1557536340848742, -300.1498634024007970 ) ) ;
#27953=CARTESIAN_POINT ( 'NONE',  ( -69.85430415644619018, -291.9805209788416391, -337.9475929042657754 ) ) ;
#27954=CARTESIAN_POINT ( 'NONE',  ( -73.44170209349182699, -291.5311599022000451, -336.1161045002704100 ) ) ;
#27955=CARTESIAN_POINT ( 'NONE',  ( -91.47367761872342840, -289.2840923547162788, -218.1358030738686580 ) ) ;
#27956=CARTESIAN_POINT ( 'NONE',  ( 24.09585832701573338, -294.9673657744388038, -227.2567852158995265 ) ) ;
#27957=CARTESIAN_POINT ( 'NONE',  ( -25.11429705045469518, -287.1530173869681448, -198.1023217635853371 ) ) ;
#27958=CARTESIAN_POINT ( 'NONE',  ( -11.80074132295477440, -294.3839197307498239, -199.6120958487989014 ) ) ;
#27961=CARTESIAN_POINT ( 'NONE',  ( -109.4702845331659518, -274.8139039863303310, -248.3680098610322204 ) ) ;
#27963=CARTESIAN_POINT ( 'NONE',  ( -92.22183984943048074, -281.8365326743239621, -321.4803014006045601 ) ) ;
#27964=CARTESIAN_POINT ( 'NONE',  ( -113.4940128995877302, -295.6160217112962982, -280.9973586397013605 ) ) ;
#27965=CARTESIAN_POINT ( 'NONE',  ( -29.86552482766319372, -272.3879355550705554, -196.7263380488801943 ) ) ;
#27966=CARTESIAN_POINT ( 'NONE',  ( -54.30538834567294515, -275.3514247613899784, -342.8956506329570288 ) ) ;
#27967=CARTESIAN_POINT ( 'NONE',  ( -72.10929422892263574, -274.7869768633194099, -205.6643640865797806 ) ) ;
#27968=CARTESIAN_POINT ( 'NONE',  ( -110.9734164504221781, -297.9626579442078764, -271.4901245234829048 ) ) ;
#27970=CARTESIAN_POINT ( 'NONE',  ( -110.5455347005672166, -297.3403183804243213, -271.4757568934718392 ) ) ;
#27972=CARTESIAN_POINT ( 'NONE',  ( 36.21379865595796588, -285.7822219247698285, -286.7905047154431486 ) ) ;
#27973=CARTESIAN_POINT ( 'NONE',  ( -110.1886153916286588, -272.4573627217373541, -264.9113385027636127 ) ) ;
#27974=CARTESIAN_POINT ( 'NONE',  ( -65.87736105605257819, -285.6890032763001273, -198.8297203755435305 ) ) ;
#27975=CARTESIAN_POINT ( 'NONE',  ( 7.535050267258309731, -286.3123054090664255, -207.7509064954122096 ) ) ;
#27976=CARTESIAN_POINT ( 'NONE',  ( -84.21346412910577328, -299.3910101241331745, -211.3573508217638448 ) ) ;
#27977=CARTESIAN_POINT ( 'NONE',  ( -66.79765748930917368, -293.4388402721720013, -339.1533777548776811 ) ) ;
#27978=CARTESIAN_POINT ( 'NONE',  ( -67.29007497460159470, -278.8664542544996721, -199.5991672970455966 ) ) ;
#27979=CARTESIAN_POINT ( 'NONE',  ( 21.27581636871891391, -291.6952119285919025, -317.1477375740089997 ) ) ;
#27981=CARTESIAN_POINT ( 'NONE',  ( -21.05608060528523851, -287.6334131177407016, -341.9286322635841202 ) ) ;
#27983=CARTESIAN_POINT ( 'NONE',  ( -28.97461484905128515, -286.9459128861973909, -344.8929402574292453 ) ) ;
#27984=CARTESIAN_POINT ( 'NONE',  ( -91.64643365806763597, -274.7806438306192831, -220.5257315113691732 ) ) ;
#27985=CARTESIAN_POINT ( 'NONE',  ( -19.90843096779035903, -281.6971225055159493, -195.9112900974531613 ) ) ;
#27986=CARTESIAN_POINT ( 'NONE',  ( -87.52917990643007329, -293.7681210646803152, -326.6416414990556518 ) ) ;
#27987=CARTESIAN_POINT ( 'NONE',  ( 18.49435572935509953, -282.2203537072990116, -317.4053548136532754 ) ) ;
#27988=CARTESIAN_POINT ( 'NONE',  ( -103.8508741773613338, -297.2248935143250037, -231.4548793782386156 ) ) ;
#27989=CARTESIAN_POINT ( 'NONE',  ( -86.57776161076688481, -298.8731386555825793, -215.5293935837487140 ) ) ;
#27990=CARTESIAN_POINT ( 'NONE',  ( -2.098379140744467186, -282.5189682755772083, -204.1575759557293281 ) ) ;
#27991=CARTESIAN_POINT ( 'NONE',  ( -94.96597827460345798, -294.9756243184080517, -315.5590274144084901 ) ) ;
#27994=CARTESIAN_POINT ( 'NONE',  ( -62.05604516651806080, -285.3548235517718012, -340.8502527955778305 ) ) ;
#27996=CARTESIAN_POINT ( 'NONE',  ( -110.4542110544635705, -288.2666405000204577, -253.6410175316879361 ) ) ;
#27997=CARTESIAN_POINT ( 'NONE',  ( 38.56968178120676782, -274.5991142934987010, -258.3757766717307618 ) ) ;
#27998=CARTESIAN_POINT ( 'NONE',  ( 12.90469444076323668, -292.6109992374461513, -217.4054777038944621 ) ) ;
#27999=CARTESIAN_POINT ( 'NONE',  ( 36.04086593327440369, -282.9769203603686947, -263.0636187760797498 ) ) ;
#28000=CARTESIAN_POINT ( 'NONE',  ( 34.90031361873190718, -276.9546506386490137, -255.2153453687832609 ) ) ;
#28001=CARTESIAN_POINT ( 'NONE',  ( -37.29624056562353474, -284.4768226468576700, -346.7848434621091656 ) ) ;
#28002=CARTESIAN_POINT ( 'NONE',  ( 35.91712305628837498, -280.2879916519581229, -265.8583044698336835 ) ) ;
#28003=CARTESIAN_POINT ( 'NONE',  ( -112.1616053369291279, -280.4765637453513136, -276.2608981042075698 ) ) ;
#28004=CARTESIAN_POINT ( 'NONE',  ( -36.89686204664280211, -298.0575775464870958, -193.3611179820811401 ) ) ;
#28005=CARTESIAN_POINT ( 'NONE',  ( 1.045191405193388823, -276.3882277681180426, -337.1707270143655819 ) ) ;
#28006=CARTESIAN_POINT ( 'NONE',  ( 34.51298934953057795, -295.7248008620028941, -289.8574664704102588 ) ) ;
#28010=CARTESIAN_POINT ( 'NONE',  ( -112.5458065890736492, -294.8086773902774098, -261.1606913031427553 ) ) ;
#28011=CARTESIAN_POINT ( 'NONE',  ( 31.17820085880634551, -274.7219550178333520, -245.0034443843609893 ) ) ;
#28013=CARTESIAN_POINT ( 'NONE',  ( 33.81202857369787296, -295.4246590639627925, -297.9265790378584029 ) ) ;
#28014=CARTESIAN_POINT ( 'NONE',  ( 31.82082319512121416, -294.3314994450817608, -237.3053287517543595 ) ) ;
#28015=CARTESIAN_POINT ( 'NONE',  ( -81.46852711905823696, -291.6536940049837767, -330.8644088861172463 ) ) ;
#28016=CARTESIAN_POINT ( 'NONE',  ( -54.39588776401409831, -275.2714312198598350, -343.2787136585802727 ) ) ;
#28017=CARTESIAN_POINT ( 'NONE',  ( -64.84282839875992011, -279.3341592742543185, -339.5895602522381296 ) ) ;
#28018=CARTESIAN_POINT ( 'NONE',  ( -42.51371024838580581, -293.1977432530407555, -344.6212318387199502 ) ) ;
#28019=CARTESIAN_POINT ( 'NONE',  ( 12.88003433711540424, -284.2207523445686093, -327.1591206434434298 ) ) ;
#28021=CARTESIAN_POINT ( 'NONE',  ( -99.86580070651493202, -283.9988228077532995, -231.9895940736992657 ) ) ;
#28022=CARTESIAN_POINT ( 'NONE',  ( 140.7777284831114173, 178.7908050832685660, -240.4635850708682199 ) ) ;
#28023=ORIENTED_EDGE ( 'NONE', *, *, #80614, .T. ) ;
#28024=CARTESIAN_POINT ( 'NONE',  ( -104.1343511845896046, -283.8218535153925473, -299.8709341718724772 ) ) ;
#28026=CARTESIAN_POINT ( 'NONE',  ( 29.01222710156249107, -282.1297269839663500, -231.9079146012832950 ) ) ;
#28027=CARTESIAN_POINT ( 'NONE',  ( -113.9582448744078391, -283.3161530564225927, -272.8210911669781922 ) ) ;
#28028=CARTESIAN_POINT ( 'NONE',  ( -95.73465106590919049, -280.1677410188584645, -220.5103765501183659 ) ) ;
#28030=CARTESIAN_POINT ( 'NONE',  ( -113.0756255427715757, -279.9492366175376787, -280.1102947509685350 ) ) ;
#28031=CARTESIAN_POINT ( 'NONE',  ( -37.30987171927208124, -297.5519495502701375, -340.3611179825599606 ) ) ;
#28032=CARTESIAN_POINT ( 'NONE',  ( 198.4579507164851009, 284.8021970988023099, -111.8421920981697468 ) ) ;
#28034=CARTESIAN_POINT ( 'NONE',  ( -110.9373293241335432, -274.7303055138964396, -256.5293980630806345 ) ) ;
#28036=CARTESIAN_POINT ( 'NONE',  ( -94.32997554917086802, -277.2425367033696944, -222.1316811135891953 ) ) ;
#28037=CARTESIAN_POINT ( 'NONE',  ( -94.90809356893018389, -292.9911176452388304, -220.7419850043174847 ) ) ;
#28038=CARTESIAN_POINT ( 'NONE',  ( 30.92654188914169922, -292.5521051785483451, -244.2203490601783358 ) ) ;
#28039=CARTESIAN_POINT ( 'NONE',  ( -46.02505861133587928, -288.6669869282663967, -346.8610871995458069 ) ) ;
#28041=CARTESIAN_POINT ( 'NONE',  ( 12.99392934457449478, -292.9403333033848185, -327.9197831423583125 ) ) ;
#28042=CARTESIAN_POINT ( 'NONE',  ( 5.203008780962274038, -285.0377962690827758, -209.9960987087968078 ) ) ;
#28043=CARTESIAN_POINT ( 'NONE',  ( -80.26387722345732811, -293.3247882169677041, -209.7295227356470377 ) ) ;
#28044=CARTESIAN_POINT ( 'NONE',  ( 31.82436773254024942, -283.1977697238015139, -295.3571764910120123 ) ) ;
#28046=CARTESIAN_POINT ( 'NONE',  ( -111.4089442134200141, -291.7473706602705761, -250.1403505333659041 ) ) ;
#28047=CARTESIAN_POINT ( 'NONE',  ( 9.311019555255182212, -281.2054999386868417, -214.0678468630394775 ) ) ;
#28048=CARTESIAN_POINT ( 'NONE',  ( 22.85009222728621481, -292.9842291068742384, -317.7631340231550325 ) ) ;
#28049=CARTESIAN_POINT ( 'NONE',  ( -40.32223792881935509, -289.8915235689477754, -347.1548679513696811 ) ) ;
#28050=CARTESIAN_POINT ( 'NONE',  ( -75.62761341090129008, -290.0412110251078275, -337.0972831956987079 ) ) ;
#28051=CARTESIAN_POINT ( 'NONE',  ( 30.48597157529096080, -288.0815754236534190, -297.4864780855438084 ) ) ;
#28054=CARTESIAN_POINT ( 'NONE',  ( -1.272993729137065877, -296.4394104881654357, -337.0042431845305373 ) ) ;
#28055=CARTESIAN_POINT ( 'NONE',  ( -112.1149302435014476, -295.4415447471848779, -254.1055185902897904 ) ) ;
#28056=CARTESIAN_POINT ( 'NONE',  ( -89.26106157956098741, -276.8634653042522586, -322.0837801763900075 ) ) ;
#28057=CARTESIAN_POINT ( 'NONE',  ( -95.03617356095902835, -272.7495893077818323, -219.4604830293382633 ) ) ;
#28058=CARTESIAN_POINT ( 'NONE',  ( -86.97105768655656277, -294.2380822046523008, -324.8371183800423410 ) ) ;
#28059=CARTESIAN_POINT ( 'NONE',  ( 23.87807793721375305, -276.7414679868615508, -228.7437702527872716 ) ) ;
#28060=CARTESIAN_POINT ( 'NONE',  ( -47.38841827234107740, -296.1627301703168769, -196.9809126923687757 ) ) ;
#28061=CARTESIAN_POINT ( 'NONE',  ( 19.14848069100017369, -295.4182486591070074, -317.2225090953092490 ) ) ;
#28062=CARTESIAN_POINT ( 'NONE',  ( -92.41384093303166480, -296.9439873335218749, -318.7479486428186988 ) ) ;
#28064=CARTESIAN_POINT ( 'NONE',  ( -14.00744866198116156, -296.3544873044916130, -342.9004391991400666 ) ) ;
#28065=CARTESIAN_POINT ( 'NONE',  ( -107.7299518214646241, -294.2085732513149310, -296.8808627079519624 ) ) ;
#28066=CARTESIAN_POINT ( 'NONE',  ( -37.26203148652085417, -298.7045363509798790, -193.4622787378366411 ) ) ;
#28067=CARTESIAN_POINT ( 'NONE',  ( 24.72565874737504643, -286.6691604813794356, -309.8961389004255693 ) ) ;
#28068=CARTESIAN_POINT ( 'NONE',  ( -106.2264664317372791, -274.9418047100177773, -240.5664689719322098 ) ) ;
#28069=CARTESIAN_POINT ( 'NONE',  ( -63.54203524777665990, -274.2119788028431344, -198.0211612311889269 ) ) ;
#28071=CARTESIAN_POINT ( 'NONE',  ( -92.76322366191756430, -297.5622419110973738, -222.7967240744494006 ) ) ;
#28073=CARTESIAN_POINT ( 'NONE',  ( -69.28850980877456323, -281.6138905431190551, -202.0988976426890531 ) ) ;
#28074=CARTESIAN_POINT ( 'NONE',  ( -19.85257429741055901, -278.9571171680595398, -195.8256322199339934 ) ) ;
#28075=CARTESIAN_POINT ( 'NONE',  ( 2.034808907305420078, -281.8880808434401501, -336.4126381976352036 ) ) ;
#28076=CARTESIAN_POINT ( 'NONE',  ( 38.82435768319805902, -274.7681843432404207, -259.7760141078702532 ) ) ;
#28077=CARTESIAN_POINT ( 'NONE',  ( 32.44849175900301219, -279.5578260653259690, -239.7707677089753702 ) ) ;
#28078=CARTESIAN_POINT ( 'NONE',  ( 11.81297834089748733, -278.7329559869243099, -213.4942030997031850 ) ) ;
#28079=CARTESIAN_POINT ( 'NONE',  ( -0.2335894197411676199, -273.1307780190336416, -206.7982915321937014 ) ) ;
#28080=CARTESIAN_POINT ( 'NONE',  ( 36.25921273462058281, -277.7382913887556128, -284.8457121460251074 ) ) ;
#28082=CARTESIAN_POINT ( 'NONE',  ( -110.6385569029122848, -295.0485713668923040, -250.1283228783588015 ) ) ;
#28083=CARTESIAN_POINT ( 'NONE',  ( -7.811030919525538074, -290.4572835550393961, -201.0192816191308793 ) ) ;
#28084=CARTESIAN_POINT ( 'NONE',  ( -16.62661434677074368, -292.3126276128176073, -196.1999069550090553 ) ) ;
#28086=CARTESIAN_POINT ( 'NONE',  ( -26.02034839420548451, -278.9084648971136176, -344.6703059690834721 ) ) ;
#28087=CARTESIAN_POINT ( 'NONE',  ( -24.22220845655590793, -272.2193692862254011, -196.4644972783399908 ) ) ;
#28089=CARTESIAN_POINT ( 'NONE',  ( 10.59821394562014163, -284.3163988261264876, -328.8332841813749496 ) ) ;
#28091=CARTESIAN_POINT ( 'NONE',  ( -57.85746960201582567, -283.7871510016461798, -198.1684539808781835 ) ) ;
#28093=CARTESIAN_POINT ( 'NONE',  ( 27.50171581107858998, -292.8142785873861840, -304.8566253971574724 ) ) ;
#28094=CARTESIAN_POINT ( 'NONE',  ( -11.57134551548542767, -284.5309734624110547, -200.7424832421526446 ) ) ;
#28096=CARTESIAN_POINT ( 'NONE',  ( -9.778035230499003916, -292.6919539700308519, -340.1124264062586349 ) ) ;
#28097=CARTESIAN_POINT ( 'NONE',  ( -99.23754676277074793, -282.4339519434785188, -315.0769286375563070 ) ) ;
#28098=CARTESIAN_POINT ( 'NONE',  ( -100.1592769896655142, -280.6817413980896845, -231.5286852455453186 ) ) ;
#28099=CARTESIAN_POINT ( 'NONE',  ( -78.32305721756537764, -286.7188482332049375, -205.6422097011765686 ) ) ;
#28100=CARTESIAN_POINT ( 'NONE',  ( 38.40341063769719199, -279.7152870788160044, -264.3070113555457397 ) ) ;
#28101=CARTESIAN_POINT ( 'NONE',  ( 15.97446700786748686, -286.8346201214483813, -220.4789939989699121 ) ) ;
#28102=CARTESIAN_POINT ( 'NONE',  ( -45.95922735717458352, -278.5886984747362476, -343.4950714331884569 ) ) ;
#28103=CARTESIAN_POINT ( 'NONE',  ( -83.09980543342778958, -278.4997163134779044, -327.5121914353359784 ) ) ;
#28104=CARTESIAN_POINT ( 'NONE',  ( -70.36858769287958637, -287.5988760299284763, -202.6290612783738538 ) ) ;
#28106=CARTESIAN_POINT ( 'NONE',  ( -33.33235367113654490, -297.9343723149041807, -193.3612275890083652 ) ) ;
#28107=CARTESIAN_POINT ( 'NONE',  ( 37.19341873245248564, -289.4687431499712602, -265.4540040888338694 ) ) ;
#28109=CARTESIAN_POINT ( 'NONE',  ( -55.56934967048406548, -285.7662352645559736, -350.3683826091709648 ) ) ;
#28111=CARTESIAN_POINT ( 'NONE',  ( -34.15480953538573061, -272.0919910463347264, -195.2620357165949088 ) ) ;
#28112=CARTESIAN_POINT ( 'NONE',  ( 36.31795925728029317, -292.1988635904641001, -289.8725248096885707 ) ) ;
#28113=CARTESIAN_POINT ( 'NONE',  ( -52.64186249299973497, -297.3585942447999173, -198.8676508325147552 ) ) ;
#28114=CARTESIAN_POINT ( 'NONE',  ( -19.66814652079286319, -287.8036951470864437, -198.8184506195497647 ) ) ;
#28115=CARTESIAN_POINT ( 'NONE',  ( -22.00602838502867087, -282.0113298568033997, -197.9014226922296587 ) ) ;
#28116=CARTESIAN_POINT ( 'NONE',  ( -17.85693358336884984, -290.2309328392287853, -344.2458265767364765 ) ) ;
#28117=CARTESIAN_POINT ( 'NONE',  ( -89.14518610396103782, -291.0781396373813550, -326.6611811480674419 ) ) ;
#28118=CARTESIAN_POINT ( 'NONE',  ( -95.82909910700773537, -285.9062825093197375, -317.3307111817943564 ) ) ;
#28119=CARTESIAN_POINT ( 'NONE',  ( -75.33435227619870034, -277.7109374176577035, -337.3354293807615818 ) ) ;
#28120=CARTESIAN_POINT ( 'NONE',  ( -39.09932026000416272, -293.1538992842187099, -345.9006769748923489 ) ) ;
#28121=CARTESIAN_POINT ( 'NONE',  ( -4.942056552631748367, -280.3004092114634318, -200.5093957366760549 ) ) ;
#28122=CARTESIAN_POINT ( 'NONE',  ( -106.5766844540482623, -274.7661600914407245, -243.4352046824957654 ) ) ;
#28123=CARTESIAN_POINT ( 'NONE',  ( 35.77081079830085031, -283.8376638359844719, -253.6410175316879361 ) ) ;
#28124=CARTESIAN_POINT ( 'NONE',  ( 38.36892465339373359, -273.8740213224252784, -276.8322312763607442 ) ) ;
#28125=DIRECTION ( 'NONE',  ( 0.000000000000000000, 1.000000000000000000, -1.224646799147353207E-16 ) ) ;
#28126=CARTESIAN_POINT ( 'NONE',  ( 20.22558858948192650, -281.6934121598234810, -315.3499578384507913 ) ) ;
#28127=CARTESIAN_POINT ( 'NONE',  ( -103.2562580389043205, -279.2449484700624112, -309.4943211881104048 ) ) ;
#28128=CARTESIAN_POINT ( 'NONE',  ( -65.81734592743688950, -299.0974448382855826, -202.5045596089376261 ) ) ;
#28129=CARTESIAN_POINT ( 'NONE',  ( -75.97789731365388377, -284.6084101304830369, -203.9669286006616460 ) ) ;
#28130=CARTESIAN_POINT ( 'NONE',  ( -95.73641430247434414, -291.6800915229406996, -315.8571982698352372 ) ) ;
#28131=CARTESIAN_POINT ( 'NONE',  ( -112.2852903574929542, -274.3299928845239606, -256.2986304240960749 ) ) ;
#28132=CARTESIAN_POINT ( 'NONE',  ( -38.36770459288386093, -275.3547103246697816, -193.8611468089742971 ) ) ;
#28134=CARTESIAN_POINT ( 'NONE',  ( -48.03033188651542673, -297.1884613269500051, -344.4797458317314636 ) ) ;
#28135=CARTESIAN_POINT ( 'NONE',  ( -45.87315631982862385, -281.1602700852100725, -344.7588222751869012 ) ) ;
#28136=CARTESIAN_POINT ( 'NONE',  ( -95.64212420531865178, -290.8980335871908096, -220.0736377485097535 ) ) ;
#28137=CARTESIAN_POINT ( 'NONE',  ( 12.66675576639619649, -272.7732058343387394, -214.8748835000687052 ) ) ;
#28138=CARTESIAN_POINT ( 'NONE',  ( -10.29715296642566535, -287.9992811074804990, -199.0656487114469257 ) ) ;
#28139=CARTESIAN_POINT ( 'NONE',  ( -79.69814407969313663, -290.3851741328182925, -210.4644847016560902 ) ) ;
#28141=CARTESIAN_POINT ( 'NONE',  ( -103.2990538180395248, -288.6197473780759992, -309.0434482503382583 ) ) ;
#28142=CARTESIAN_POINT ( 'NONE',  ( -81.73853767321745067, -291.0954685806805173, -212.3229330168005333 ) ) ;
#28144=CARTESIAN_POINT ( 'NONE',  ( 34.55962938336060120, -288.2931712937298130, -243.6835745483854794 ) ) ;
#28145=CARTESIAN_POINT ( 'NONE',  ( 5.412601320327937948, -276.7890038939988244, -329.6194828118274245 ) ) ;
#28146=CARTESIAN_POINT ( 'NONE',  ( 0.3764463079797041867, -293.4822351244868059, -337.1507359201993381 ) ) ;
#28147=CARTESIAN_POINT ( 'NONE',  ( -21.73855640299023406, -283.5086081065511507, -345.6595554973395110 ) ) ;
#28148=CARTESIAN_POINT ( 'NONE',  ( -46.50719114211967309, -286.2721241826269534, -193.9298543141706546 ) ) ;
#28149=CARTESIAN_POINT ( 'NONE',  ( 26.87565952756503762, -282.3595616613027914, -305.1205513143564190 ) ) ;
#28150=CARTESIAN_POINT ( 'NONE',  ( 25.26796030052132025, -22.82892349226261075, -345.1428209926129966 ) ) ;
#28151=CARTESIAN_POINT ( 'NONE',  ( -57.31220355042948000, -168.7168211105807529, -363.3665416233598648 ) ) ;
#28152=CARTESIAN_POINT ( 'NONE',  ( 83.65573564170013299, 82.10386166810425834, -298.8792467998813436 ) ) ;
#28153=CARTESIAN_POINT ( 'NONE',  ( -40.77230168148079770, -273.2052034312633282, -197.2303059850570151 ) ) ;
#28154=CARTESIAN_POINT ( 'NONE',  ( 34.13822505986901490, -274.2580367448811671, -254.0308445503238772 ) ) ;
#28155=CARTESIAN_POINT ( 'NONE',  ( -90.67393958100727502, -295.2912265906286393, -325.8889516326451030 ) ) ;
#28156=CARTESIAN_POINT ( 'NONE',  ( -81.85735553743283788, -219.3983098388335691, -349.3051352687708686 ) ) ;
#28157=CARTESIAN_POINT ( 'NONE',  ( -18.65411271695536044, -272.9726401196645043, -196.1170019598329475 ) ) ;
#28158=CARTESIAN_POINT ( 'NONE',  ( -109.7922860182429048, -298.2026840404762424, -286.5406757052586499 ) ) ;
#28159=CARTESIAN_POINT ( 'NONE',  ( -39.95886001895915030, -290.4007690617337971, -343.8575672787906683 ) ) ;
#28160=CARTESIAN_POINT ( 'NONE',  ( -108.4115248816573001, -291.8687437960538773, -252.3293109300332446 ) ) ;
#28162=CARTESIAN_POINT ( 'NONE',  ( -51.76818457096969439, -298.8132971490065870, -194.9100150582193010 ) ) ;
#28164=CARTESIAN_POINT ( 'NONE',  ( -0.9553561296519736956, -289.0478212563090779, -333.7756677901251123 ) ) ;
#28165=CARTESIAN_POINT ( 'NONE',  ( 23.90646584971814192, -294.9744124262732043, -316.7596199564286508 ) ) ;
#28166=CARTESIAN_POINT ( 'NONE',  ( -0.7299311085422596213, -295.0715627795631235, -338.0450784592586047 ) ) ;
#28167=CARTESIAN_POINT ( 'NONE',  ( 29.49090886667639921, -294.1139096438990350, -299.7278062438883239 ) ) ;
#28169=CARTESIAN_POINT ( 'NONE',  ( 15.95714609906237058, -278.2245376995158495, -323.9930235821350379 ) ) ;
#28171=CARTESIAN_POINT ( 'NONE',  ( -79.87153957028512252, -279.0016068032708176, -206.1821622566758379 ) ) ;
#28172=CARTESIAN_POINT ( 'NONE',  ( 35.61146836546884487, -276.4016974978463850, -263.3864527957813380 ) ) ;
#28173=CARTESIAN_POINT ( 'NONE',  ( -43.97691090012794035, -275.7296400576510678, -194.6120907048616289 ) ) ;
#28174=CARTESIAN_POINT ( 'NONE',  ( 29.08106880941043215, -274.0435382624835938, -306.0580591023386887 ) ) ;
#28175=CARTESIAN_POINT ( 'NONE',  ( -107.9362574306327929, -297.4545039448234434, -251.3312609251844947 ) ) ;
#28176=CARTESIAN_POINT ( 'NONE',  ( -101.9935680215305212, -294.6509622677120319, -305.5109528833190211 ) ) ;
#28177=CARTESIAN_POINT ( 'NONE',  ( 144.2857639756989272, -299.5541904835127980, -202.0153591320744226 ) ) ;
#28178=CARTESIAN_POINT ( 'NONE',  ( -114.3163711564752134, -279.0647664114617896, -268.7418033755333795 ) ) ;
#28180=CARTESIAN_POINT ( 'NONE',  ( -6.274698393131096452, -276.7989492697439005, -336.4342645810056638 ) ) ;
#28181=CARTESIAN_POINT ( 'NONE',  ( 28.28420850146423859, -285.7196752927730472, -230.9328562144431771 ) ) ;
#28182=CARTESIAN_POINT ( 'NONE',  ( -112.3417001280813992, -274.5519907608264134, -270.3865269787834222 ) ) ;
#28184=CARTESIAN_POINT ( 'NONE',  ( 32.43066532167586757, -286.4577060278090244, -248.3096427053020818 ) ) ;
#28185=CARTESIAN_POINT ( 'NONE',  ( -24.68131805288838265, -278.4557568257499156, -197.4386335419287093 ) ) ;
#28186=CARTESIAN_POINT ( 'NONE',  ( -107.7859579568138173, -277.4064100955260983, -249.0777569567908358 ) ) ;
#28187=CARTESIAN_POINT ( 'NONE',  ( -89.23430503325336360, -285.7820398157825821, -324.5815481743356372 ) ) ;
#28188=CARTESIAN_POINT ( 'NONE',  ( -43.22369394126268816, -278.3331605554121211, -343.5221229904959728 ) ) ;
#28190=CARTESIAN_POINT ( 'NONE',  ( -8.293032212393173452, -274.9168698057608822, -340.5902317083035200 ) ) ;
#28191=CARTESIAN_POINT ( 'NONE',  ( -43.49896903086576572, -274.6238782417506741, -197.4681732426494136 ) ) ;
#28192=CARTESIAN_POINT ( 'NONE',  ( 35.77123290750189000, -283.7765328698089320, -287.8668151835400977 ) ) ;
#28194=CARTESIAN_POINT ( 'NONE',  ( 37.91545077661244534, -289.5584402653669827, -277.1194782840451012 ) ) ;
#28196=CARTESIAN_POINT ( 'NONE',  ( -48.22273983581821710, -289.9136607298749482, -196.1027513855873394 ) ) ;
#28198=CARTESIAN_POINT ( 'NONE',  ( 21.08370160627710987, -273.6139865770130655, -225.7565898271020046 ) ) ;
#28199=CARTESIAN_POINT ( 'NONE',  ( 36.85665640478975291, -291.6613916260426436, -268.0224505403757576 ) ) ;
#28200=CARTESIAN_POINT ( 'NONE',  ( 28.92138380700103895, -24.05900251067409457, -347.7894294321414463 ) ) ;
#28202=CARTESIAN_POINT ( 'NONE',  ( -91.12372321394828134, -288.2790271934700286, -324.5668051599027990 ) ) ;
#28203=CARTESIAN_POINT ( 'NONE',  ( -70.55692872783261294, -285.0977153088188061, -336.2781237141655879 ) ) ;
#28204=CARTESIAN_POINT ( 'NONE',  ( 36.51413064112026774, -286.0191328881043660, -288.2847123187141278 ) ) ;
#28205=CARTESIAN_POINT ( 'NONE',  ( -64.25409643154559092, -284.8356200401500473, -338.8527075587416562 ) ) ;
#28206=CARTESIAN_POINT ( 'NONE',  ( -69.06996289883772988, -284.2832992851155609, -336.2985353886234634 ) ) ;
#28207=CARTESIAN_POINT ( 'NONE',  ( -37.81064810741841598, -294.0261927356572187, -195.0073729177867108 ) ) ;
#28208=CARTESIAN_POINT ( 'NONE',  ( 28.70103266055255276, -273.1458537488143179, -233.5428177046572387 ) ) ;
#28209=CARTESIAN_POINT ( 'NONE',  ( -1.315148466027089347, -274.8500468257770990, -202.3329483252103103 ) ) ;
#28210=CARTESIAN_POINT ( 'NONE',  ( -111.4603495875456218, -288.4439694074263230, -285.1148957839625950 ) ) ;
#28211=CARTESIAN_POINT ( 'NONE',  ( -77.81490168422480735, -277.5794856372182835, -335.9281926935486808 ) ) ;
#28212=CARTESIAN_POINT ( 'NONE',  ( 28.62316312046310429, -295.9987339488381508, -305.4070589946056202 ) ) ;
#28214=CARTESIAN_POINT ( 'NONE',  ( -4.771743288812468897, -297.1233781216987495, -337.9199732462171255 ) ) ;
#28215=CARTESIAN_POINT ( 'NONE',  ( -94.68021586434736037, -282.5914848497494063, -316.3543759677571643 ) ) ;
#28216=CARTESIAN_POINT ( 'NONE',  ( -9.577188976701833667, -278.4147702638450141, -200.6895127905459901 ) ) ;
#28218=CARTESIAN_POINT ( 'NONE',  ( -102.1201425696595919, -271.5644569664745518, -230.0317100195215971 ) ) ;
#28219=CARTESIAN_POINT ( 'NONE',  ( -76.41730650169333217, -276.9381154945092476, -332.2024458730276137 ) ) ;
#28220=CARTESIAN_POINT ( 'NONE',  ( 29.35789448925144995, -294.6515473460921157, -238.9059162442042634 ) ) ;
#28221=CARTESIAN_POINT ( 'NONE',  ( 16.90442126109993737, -293.7899599567780342, -221.0854665434989670 ) ) ;
#28222=CARTESIAN_POINT ( 'NONE',  ( -53.17075368909969058, -296.5660545582534837, -345.2667576224077948 ) ) ;
#28223=CARTESIAN_POINT ( 'NONE',  ( -109.1425161710217679, -296.2107265850891622, -283.6077357180204785 ) ) ;
#28224=CARTESIAN_POINT ( 'NONE',  ( -28.92403570801938528, -290.9455890375159584, -344.8872447663294452 ) ) ;
#28225=CARTESIAN_POINT ( 'NONE',  ( -113.4877514638859992, -284.8662507383784259, -258.5736007833649523 ) ) ;
#28226=CARTESIAN_POINT ( 'NONE',  ( 11.01583020941407121, -272.8523817500299060, -211.9675058205340008 ) ) ;
#28227=CARTESIAN_POINT ( 'NONE',  ( 27.13891865678215254, -286.8325718297650724, -228.2748992687869247 ) ) ;
#28228=CARTESIAN_POINT ( 'NONE',  ( -60.26213215570052739, -281.7335712239016061, -199.2678796310722475 ) ) ;
#28229=CARTESIAN_POINT ( 'NONE',  ( -96.75872625015618667, -284.2079516786839690, -227.5258824215704578 ) ) ;
#28230=CARTESIAN_POINT ( 'NONE',  ( -73.48640904561523257, -287.5314850700121383, -336.0915394860306264 ) ) ;
#28231=CARTESIAN_POINT ( 'NONE',  ( 126.6218730542261568, 145.9178657400643431, -262.1768218896158373 ) ) ;
#28232=CARTESIAN_POINT ( 'NONE',  ( 20.39313511829428904, -286.4297090199575564, -225.5874958269120043 ) ) ;
#28233=CARTESIAN_POINT ( 'NONE',  ( -27.39068880348714785, -283.8700397890278282, -346.5313159530292069 ) ) ;
#28234=CARTESIAN_POINT ( 'NONE',  ( -104.3985991894187464, -290.0968076811613514, -232.9954586059634494 ) ) ;
#28236=CARTESIAN_POINT ( 'NONE',  ( -97.95254533299885225, -280.7745758153931206, -224.1579778351505468 ) ) ;
#28237=CARTESIAN_POINT ( 'NONE',  ( -73.54714586137188803, -280.8972150909823426, -202.9484576090193855 ) ) ;
#28238=CARTESIAN_POINT ( 'NONE',  ( 18.83746333747442137, -280.7241845885035900, -223.7273239982240511 ) ) ;
#28239=CARTESIAN_POINT ( 'NONE',  ( 22.25570254758597244, -276.9287847461008596, -224.8081276612231534 ) ) ;
#28240=CARTESIAN_POINT ( 'NONE',  ( -65.60349775875658906, -295.4116592975155413, -342.0012486326589851 ) ) ;
#28241=CARTESIAN_POINT ( 'NONE',  ( 17.19584324582809032, -286.2898704726347887, -321.4024250702861423 ) ) ;
#28242=CARTESIAN_POINT ( 'NONE',  ( 10.59948876026856013, -294.3015937381687195, -211.0641761292658316 ) ) ;
#28243=CARTESIAN_POINT ( 'NONE',  ( -97.12689406063604736, -296.0624191245326529, -227.9352218751724308 ) ) ;
#28244=EDGE_LOOP ( 'NONE', ( #63106, #24772, #62377, #26872, #39608 ) ) ;
#28245=CARTESIAN_POINT ( 'NONE',  ( -33.39591625071374636, -284.9222791111476454, -344.7092933470706271 ) ) ;
#28246=CARTESIAN_POINT ( 'NONE',  ( -109.3844692818184114, -296.0617587240714670, -282.2744256454533343 ) ) ;
#28247=CARTESIAN_POINT ( 'NONE',  ( 6.308962904953159700, -293.7095395394031812, -207.3046978034235792 ) ) ;
#28248=CARTESIAN_POINT ( 'NONE',  ( 7.863494910495058221, -283.0675139387952299, -327.8747319127886612 ) ) ;
#28249=CARTESIAN_POINT ( 'NONE',  ( -58.04659286304920585, -272.8498895435625400, -196.3861271410816585 ) ) ;
#28250=CARTESIAN_POINT ( 'NONE',  ( -75.60575182150422791, -290.2002513685679901, -337.0632553892853593 ) ) ;
#28251=CARTESIAN_POINT ( 'NONE',  ( -13.82813477853880180, -280.8897849415487258, -342.3848482620905997 ) ) ;
#28252=CARTESIAN_POINT ( 'NONE',  ( -111.9004935473823252, -290.6451154730147550, -289.5640506319537053 ) ) ;
#28253=CARTESIAN_POINT ( 'NONE',  ( -26.46755010455341051, -289.2433848408505810, -342.6191097243445256 ) ) ;
#28256=CARTESIAN_POINT ( 'NONE',  ( 193.2925842856977283, 275.7319325034035273, -124.0216442356983322 ) ) ;
#28257=CARTESIAN_POINT ( 'NONE',  ( -106.6379572354042296, -270.4809262143061233, -236.9535640164627353 ) ) ;
#28258=CARTESIAN_POINT ( 'NONE',  ( -109.6532155393864798, -277.6029532917806364, -281.4807612333127622 ) ) ;
#28260=CARTESIAN_POINT ( 'NONE',  ( -68.64285039021375212, -278.5510994786062611, -204.0703639745659927 ) ) ;
#28261=CARTESIAN_POINT ( 'NONE',  ( 38.70738402024316116, -275.0685898997495542, -258.3479583630651746 ) ) ;
#28262=CARTESIAN_POINT ( 'NONE',  ( 190.8835322504810676, 268.3746148070026152, -138.2713062114818285 ) ) ;
#28263=CARTESIAN_POINT ( 'NONE',  ( -45.19462286533578776, -278.5294077734797042, -194.3023633270605615 ) ) ;
#28264=CARTESIAN_POINT ( 'NONE',  ( -104.5033528016349464, -282.1396040418259190, -303.0553471374125252 ) ) ;
#28265=CARTESIAN_POINT ( 'NONE',  ( -111.8988365848795041, -298.4990520223184376, -255.6241553476149591 ) ) ;
#28266=CARTESIAN_POINT ( 'NONE',  ( 34.00854564896192045, -293.8365349737172210, -254.5828940317004196 ) ) ;
#28268=CARTESIAN_POINT ( 'NONE',  ( -110.8606930591889324, -289.2622454714943956, -268.4322173840665187 ) ) ;
#28269=CARTESIAN_POINT ( 'NONE',  ( -27.01842774447975870, -274.8313914881420601, -194.1057720772648736 ) ) ;
#28270=CARTESIAN_POINT ( 'NONE',  ( -47.27484840216956741, -298.0892411032280620, -197.9888690110764458 ) ) ;
#28275=CARTESIAN_POINT ( 'NONE',  ( 2.862065401724003699, -281.6850157889714978, -208.9986366600172403 ) ) ;
#28276=CARTESIAN_POINT ( 'NONE',  ( 10.17168953740782378, -282.4568323180754419, -210.9940145562682687 ) ) ;
#28277=CARTESIAN_POINT ( 'NONE',  ( -106.7514822109890105, -283.9220947784536975, -246.8423828427566775 ) ) ;
#28278=CARTESIAN_POINT ( 'NONE',  ( -1.388249863805268713, -282.3947712243137858, -205.4133320649779364 ) ) ;
#28279=CARTESIAN_POINT ( 'NONE',  ( -3.566783299242565430, -275.0777469910586888, -335.8589251771521731 ) ) ;
#28280=DIRECTION ( 'NONE',  ( -1.000000000000000000, -0.000000000000000000, -0.000000000000000000 ) ) ;
#28281=CARTESIAN_POINT ( 'NONE',  ( -37.11715091922809506, -277.8522009983414023, -347.2123456663356933 ) ) ;
#28285=CARTESIAN_POINT ( 'NONE',  ( -107.7567829909006178, -286.1832625031181578, -297.3414952590535449 ) ) ;
#28286=CARTESIAN_POINT ( 'NONE',  ( 24.99079450515892020, -292.2213257825347910, -231.9600675560892000 ) ) ;
#28288=CARTESIAN_POINT ( 'NONE',  ( -14.98981534668951454, -288.1187496797799668, -343.9946843718208243 ) ) ;
#28289=CARTESIAN_POINT ( 'NONE',  ( -35.89144408075565451, -284.3104467680829543, -196.3619911400743945 ) ) ;
#28290=CARTESIAN_POINT ( 'NONE',  ( -62.74941192218881980, -284.2897048478316151, -201.2428744651817851 ) ) ;
#28291=CARTESIAN_POINT ( 'NONE',  ( -12.97512089154715653, -286.9709733649725649, -340.2484832851479837 ) ) ;
#28292=CARTESIAN_POINT ( 'NONE',  ( 14.21446335635532954, -283.5134547372127258, -322.6734096486179055 ) ) ;
#28293=CARTESIAN_POINT ( 'NONE',  ( -8.437187426262960699, -272.4302129329582272, -201.0995521608556089 ) ) ;
#28294=CARTESIAN_POINT ( 'NONE',  ( -84.99657131749313521, -283.8068220410114009, -210.9014369767490393 ) ) ;
#28295=CARTESIAN_POINT ( 'NONE',  ( -41.80051706656752941, -297.1083613085517641, -345.2794979898001770 ) ) ;
#28296=CARTESIAN_POINT ( 'NONE',  ( -111.9957770044708383, -282.6642618403684537, -261.5977150279383636 ) ) ;
#28297=CARTESIAN_POINT ( 'NONE',  ( -99.67427751751634446, -280.0229711684557969, -231.8188253953773597 ) ) ;
#28298=CARTESIAN_POINT ( 'NONE',  ( 4.146041451738739170, -288.6095584392433011, -207.6190294715171660 ) ) ;
#28301=CARTESIAN_POINT ( 'NONE',  ( 37.79147270589700724, -295.3640016885484556, -261.8631178182608323 ) ) ;
#28302=CARTESIAN_POINT ( 'NONE',  ( -111.9530736642375501, -276.6562656018784310, -262.2398140564039295 ) ) ;
#28303=CARTESIAN_POINT ( 'NONE',  ( -114.2070411641225576, -289.7745416608204323, -268.3487175639312454 ) ) ;
#28304=CARTESIAN_POINT ( 'NONE',  ( -5.211432686409379400, -293.0219433526013972, -336.8136683314594393 ) ) ;
#28305=CARTESIAN_POINT ( 'NONE',  ( 2.988507873670241732, -279.2905561233907861, -208.8613125284154250 ) ) ;
#28306=CARTESIAN_POINT ( 'NONE',  ( -111.7807899796114839, -270.6682393416608079, -267.5591356020806870 ) ) ;
#28308=CARTESIAN_POINT ( 'NONE',  ( -92.05139610758976687, -292.5650613949779881, -221.2699691272126472 ) ) ;
#28309=CARTESIAN_POINT ( 'NONE',  ( -37.37352853689063892, -276.5519495502701943, -195.3611179825600175 ) ) ;
#28310=CARTESIAN_POINT ( 'NONE',  ( -22.25374103378196011, -293.3421642802720726, -345.1612599696929919 ) ) ;
#28311=CARTESIAN_POINT ( 'NONE',  ( 24.18762060913717704, -289.7118520561572836, -311.1344624296644383 ) ) ;
#28312=CARTESIAN_POINT ( 'NONE',  ( -22.37120057738430390, -290.4810262123950224, -195.8101340056990978 ) ) ;
#28313=CARTESIAN_POINT ( 'NONE',  ( -48.12957299507327491, -290.6172278044049335, -343.2067586893828093 ) ) ;
#28315=CARTESIAN_POINT ( 'NONE',  ( -10.65569201325464910, -289.4979349682825500, -338.5363695234173633 ) ) ;
#28317=CARTESIAN_POINT ( 'NONE',  ( -98.70181860357061510, -291.1436925374194402, -316.2406777845557144 ) ) ;
#28318=CARTESIAN_POINT ( 'NONE',  ( 23.28379039339642986, -278.9645514771179364, -225.6067136813653065 ) ) ;
#28319=CARTESIAN_POINT ( 'NONE',  ( -109.7895141777525367, -290.4339308599354581, -279.3229391939135553 ) ) ;
#28320=CARTESIAN_POINT ( 'NONE',  ( -41.01163423075385595, -280.3404657819189083, -193.4566010151165472 ) ) ;
#28321=CARTESIAN_POINT ( 'NONE',  ( 38.84973329861187352, -281.3562580944006299, -281.3433656533117642 ) ) ;
#28322=CARTESIAN_POINT ( 'NONE',  ( 34.21430011340099497, -285.8438185006478989, -293.0001849796011015 ) ) ;
#28324=CARTESIAN_POINT ( 'NONE',  ( 29.24876831152463197, -280.1303457736433984, -303.2889034600283935 ) ) ;
#28325=CARTESIAN_POINT ( 'NONE',  ( -63.81672455304082803, -283.7068214046984167, -200.1755758578940174 ) ) ;
#28327=CARTESIAN_POINT ( 'NONE',  ( -113.3898918052547202, -276.9451060890970098, -277.2490561028980096 ) ) ;
#28328=CARTESIAN_POINT ( 'NONE',  ( -7.450868010730220092, -285.3551958583295800, -199.6786931537127145 ) ) ;
#28329=CARTESIAN_POINT ( 'NONE',  ( -14.02363297095190653, -275.1653942578785177, -201.0151053300785406 ) ) ;
#28331=CARTESIAN_POINT ( 'NONE',  ( -41.65979929593486020, -293.5971313076430533, -196.6371591474400589 ) ) ;
#28332=CARTESIAN_POINT ( 'NONE',  ( -35.55589187825142972, -275.4993826257528440, -193.9581857035290113 ) ) ;
#28333=CARTESIAN_POINT ( 'NONE',  ( -76.37070613831363630, -277.2561962624366174, -332.1362596562551630 ) ) ;
#28334=CARTESIAN_POINT ( 'NONE',  ( -110.4315724295534693, -291.0256432409331637, -245.9688349423528848 ) ) ;
#28335=CARTESIAN_POINT ( 'NONE',  ( 31.86402919032397563, -279.2378518939059973, -240.0315742205260676 ) ) ;
#28336=CARTESIAN_POINT ( 'NONE',  ( -7.188246166747680910, -292.2702027453557321, -199.4964663984306128 ) ) ;
#28337=CARTESIAN_POINT ( 'NONE',  ( -60.32146125780350587, -290.8056370598891363, -200.7713084256891705 ) ) ;
#28338=CARTESIAN_POINT ( 'NONE',  ( -22.51840680678187567, -292.8622030125993092, -343.8816635520170735 ) ) ;
#28341=CARTESIAN_POINT ( 'NONE',  ( 22.64203867691799132, -292.4786581677000186, -228.6264896721686171 ) ) ;
#28343=CARTESIAN_POINT ( 'NONE',  ( -6.998514795304330072, -280.1237833571632336, -333.4427485647536855 ) ) ;
#28344=CARTESIAN_POINT ( 'NONE',  ( -97.23142217410500621, -294.9653202116670059, -318.4031849749455318 ) ) ;
#28345=CARTESIAN_POINT ( 'NONE',  ( -106.2423027022131095, -286.2967567186024098, -237.1044609596501687 ) ) ;
#28346=CARTESIAN_POINT ( 'NONE',  ( 29.96259376634963800, -287.0045857113311172, -241.9612783996791165 ) ) ;
#28347=CARTESIAN_POINT ( 'NONE',  ( 10.12527082571453718, -277.9037474629217854, -326.7312733756273815 ) ) ;
#28348=CARTESIAN_POINT ( 'NONE',  ( 36.93462677629541702, -291.4702222292804663, -262.4521460158393893 ) ) ;
#28349=CARTESIAN_POINT ( 'NONE',  ( -63.91212782299929529, -297.1634670437745740, -339.4949773434000804 ) ) ;
#28350=CARTESIAN_POINT ( 'NONE',  ( -29.68719177125014852, -275.7481403152637540, -343.4091425660722621 ) ) ;
#28353=CARTESIAN_POINT ( 'NONE',  ( -68.22159410805548418, -295.1134861140318435, -340.8747793495459177 ) ) ;
#28354=CARTESIAN_POINT ( 'NONE',  ( -31.73904115706336526, -290.9011888229114220, -344.6416052184358136 ) ) ;
#28355=CARTESIAN_POINT ( 'NONE',  ( -77.68490200995596240, -295.5107798038987426, -207.0751259330633332 ) ) ;
#28356=CARTESIAN_POINT ( 'NONE',  ( -26.45152270995227894, -289.5614656518309857, -342.6984529841714675 ) ) ;
#28358=CARTESIAN_POINT ( 'NONE',  ( 19.96105889002106437, -279.9160973750380208, -219.2608830957678947 ) ) ;
#28359=CARTESIAN_POINT ( 'NONE',  ( 11.14048502495207593, -295.0526103053552447, -330.1188594882695497 ) ) ;
#28360=CARTESIAN_POINT ( 'NONE',  ( -67.58297230049872439, -287.5842880753826307, -339.8288870556209531 ) ) ;
#28361=CARTESIAN_POINT ( 'NONE',  ( -92.67885520298236202, -296.1521376562493515, -323.8732059600917523 ) ) ;
#28362=CARTESIAN_POINT ( 'NONE',  ( 19.71294465489122771, -294.5291887324432878, -315.9535769871431512 ) ) ;
#28366=CARTESIAN_POINT ( 'NONE',  ( 38.66220832902902060, -288.9794338081946421, -263.0046742499005177 ) ) ;
#28367=CARTESIAN_POINT ( 'NONE',  ( -55.63300648810263738, -282.3376638359844151, -190.3683826091709363 ) ) ;
#28368=CARTESIAN_POINT ( 'NONE',  ( -69.91164440902817034, -278.9830115240158079, -200.6867775767822479 ) ) ;
#28369=CARTESIAN_POINT ( 'NONE',  ( -51.33638705727141627, -285.2315219397586361, -343.9270957213098541 ) ) ;
#28370=CARTESIAN_POINT ( 'NONE',  ( 29.62398548833278156, -285.6453926094040412, -233.4517842346842258 ) ) ;
#28372=CARTESIAN_POINT ( 'NONE',  ( 37.06829794255180843, -285.6771417894561296, -273.8512573091762192 ) ) ;
#28373=CARTESIAN_POINT ( 'NONE',  ( 36.97547293525119727, -277.5999108600984187, -285.1009711396022794 ) ) ;
#28375=CARTESIAN_POINT ( 'NONE',  ( -107.2271173388270284, -278.8314523100888778, -249.2654202865838613 ) ) ;
#28376=CARTESIAN_POINT ( 'NONE',  ( -110.2597366796839395, -277.9689982681035190, -265.1791672499649621 ) ) ;
#28377=CARTESIAN_POINT ( 'NONE',  ( -35.54486669291351575, -275.1538376283556318, -193.6782033881368363 ) ) ;
#28378=CARTESIAN_POINT ( 'NONE',  ( -77.27236899099928280, -278.3246323492271586, -204.9273191779148533 ) ) ;
#28379=CARTESIAN_POINT ( 'NONE',  ( -109.8935430929009840, -264.1146777768358334, -305.7921915240701196 ) ) ;
#28380=CARTESIAN_POINT ( 'NONE',  ( -112.8391045486285975, -273.6712229691746643, -256.1860008254682270 ) ) ;
#28381=CARTESIAN_POINT ( 'NONE',  ( -3.751190591230367133, -299.8901968535543574, -193.9423814121325620 ) ) ;
#28383=CARTESIAN_POINT ( 'NONE',  ( -106.6662871844225293, -293.4805209788415823, -237.0123917617630980 ) ) ;
#28385=DIRECTION ( 'NONE',  ( 0.000000000000000000, 0.000000000000000000, 1.000000000000000000 ) ) ;
#28386=CARTESIAN_POINT ( 'NONE',  ( -83.85456148404830401, -286.4759049093451608, -213.6314077734191130 ) ) ;
#28387=CARTESIAN_POINT ( 'NONE',  ( -109.0287915748000245, -286.6343918355893834, -245.1632027404195640 ) ) ;
#28388=CARTESIAN_POINT ( 'NONE',  ( 14.14930715884026569, -287.6537511809348757, -322.2510865376845572 ) ) ;
#28389=CARTESIAN_POINT ( 'NONE',  ( -103.9840160314192730, -284.5612455575871422, -231.8061457548824080 ) ) ;
#28390=CARTESIAN_POINT ( 'NONE',  ( -66.36576111139123668, -278.0655631838487238, -202.4942231890591131 ) ) ;
#28391=CARTESIAN_POINT ( 'NONE',  ( -11.61577298641283562, -288.2512052509643468, -200.7260538792021123 ) ) ;
#28392=CARTESIAN_POINT ( 'NONE',  ( 30.97005544243717523, -280.3987505263974072, -298.0054989999449049 ) ) ;
#28393=CARTESIAN_POINT ( 'NONE',  ( -103.5681841008370583, -279.4377183200045351, -302.3425322013466143 ) ) ;
#28394=CARTESIAN_POINT ( 'NONE',  ( 34.43278222750208784, -275.8645433489803622, -256.7078354323108442 ) ) ;
#28395=CARTESIAN_POINT ( 'NONE',  ( -23.39935020333249227, -287.6727716158931116, -345.7383852058756020 ) ) ;
#28396=CARTESIAN_POINT ( 'NONE',  ( 25.80347286089903491, -282.9348127611646078, -314.1660620642208528 ) ) ;
#28397=CARTESIAN_POINT ( 'NONE',  ( -81.52108806444685740, -284.1276142721295059, -333.4156786522270863 ) ) ;
#28398=CARTESIAN_POINT ( 'NONE',  ( -8.001393944992623020, -280.6142058573529994, -203.5032505283305682 ) ) ;
#28402=CARTESIAN_POINT ( 'NONE',  ( -2.349792472082426809, -290.4545249669257032, -337.5613551967477974 ) ) ;
#28403=CARTESIAN_POINT ( 'NONE',  ( -100.2844703387150531, -288.6589451961174859, -313.8525648565666870 ) ) ;
#28404=CARTESIAN_POINT ( 'NONE',  ( -65.89386147549961947, -272.7279132680730527, -202.9209034889935594 ) ) ;
#28406=CARTESIAN_POINT ( 'NONE',  ( 28.01490804648733146, -293.4324977709014775, -310.9806000076931127 ) ) ;
#28407=CARTESIAN_POINT ( 'NONE',  ( -56.26210232422564417, -287.7800955951983610, -341.6372508704704956 ) ) ;
#28408=CARTESIAN_POINT ( 'NONE',  ( 35.48422810754055945, -291.6192854011053441, -257.0860523830502302 ) ) ;
#28409=CARTESIAN_POINT ( 'NONE',  ( 23.85670293687120846, -288.1969690799986665, -229.7489374369895074 ) ) ;
#28410=CARTESIAN_POINT ( 'NONE',  ( -106.6662871844225293, -287.4805209788416391, -237.0123917617630980 ) ) ;
#28411=CARTESIAN_POINT ( 'NONE',  ( -15.50945203929048866, -290.7698964510578321, -342.1674554648361095 ) ) ;
#28412=CARTESIAN_POINT ( 'NONE',  ( -40.52857529660360569, -290.0120326590459285, -195.2491665500594706 ) ) ;
#28413=CARTESIAN_POINT ( 'NONE',  ( -109.7767041371149332, -292.8028757421384398, -250.8657049353424497 ) ) ;
#28414=CARTESIAN_POINT ( 'NONE',  ( -96.10339076390474133, -284.8822623916798875, -314.0700662918847001 ) ) ;
#28415=CARTESIAN_POINT ( 'NONE',  ( -9.221295223462485424, -294.4191020264000258, -200.6526446415019791 ) ) ;
#28418=CARTESIAN_POINT ( 'NONE',  ( -52.24552229563639827, -275.8422797947567915, -196.4411800919441760 ) ) ;
#28419=CARTESIAN_POINT ( 'NONE',  ( 17.71965796332989740, -281.4351889464814462, -318.5363042554145636 ) ) ;
#28420=CARTESIAN_POINT ( 'NONE',  ( -86.18299073586358361, -281.7294940876061560, -327.2779782051489406 ) ) ;
#28421=CARTESIAN_POINT ( 'NONE',  ( -70.74693375525615124, -294.6786811575623801, -339.5727745412522154 ) ) ;
#28422=CARTESIAN_POINT ( 'NONE',  ( -57.11101232590282706, -272.0336020947864313, -198.9834266358783452 ) ) ;
#28423=CARTESIAN_POINT ( 'NONE',  ( -69.90294619096133033, -275.5641426381071710, -337.3160951345850549 ) ) ;
#28424=CARTESIAN_POINT ( 'NONE',  ( -108.0729060057444428, -297.6052626141399742, -290.3195746836731814 ) ) ;
#28425=CARTESIAN_POINT ( 'NONE',  ( -53.25928572453645415, -296.6854281607849089, -342.2606168857566331 ) ) ;
#28427=CARTESIAN_POINT ( 'NONE',  ( -10.42109369833701038, -295.4944946105301824, -338.3896610843711983 ) ) ;
#28428=CARTESIAN_POINT ( 'NONE',  ( -2.950580946930152937, -284.5243794501732850, -203.2970123157070361 ) ) ;
#28429=CARTESIAN_POINT ( 'NONE',  ( -75.21064462323710131, -297.5325194028824285, -207.8930324880744251 ) ) ;
#28430=CARTESIAN_POINT ( 'NONE',  ( -73.61301432528566124, -285.5847271407538983, -202.3801102728685350 ) ) ;
#28431=CARTESIAN_POINT ( 'NONE',  ( 39.06903997543155072, -287.3410128355357074, -280.1247140277017706 ) ) ;
#28432=CARTESIAN_POINT ( 'NONE',  ( -39.04483975007040186, -297.0533146916417877, -345.6970730218347398 ) ) ;
#28433=CARTESIAN_POINT ( 'NONE',  ( -9.010354017486729816, -290.4232240499913473, -201.0429720676251009 ) ) ;
#28434=CARTESIAN_POINT ( 'NONE',  ( -74.92002003295255008, -278.7619707004824932, -203.3385196015004794 ) ) ;
#28435=CARTESIAN_POINT ( 'NONE',  ( 10.64812456238590599, -284.1952119285918457, -210.2361428286349394 ) ) ;
#28437=CARTESIAN_POINT ( 'NONE',  ( -19.70566616733899323, -285.0789360147833804, -199.1143579876925003 ) ) ;
#28439=CARTESIAN_POINT ( 'NONE',  ( 9.201713644166414241, -286.4127103764753315, -329.1719271935503457 ) ) ;
#28440=CARTESIAN_POINT ( 'NONE',  ( -75.64307371856145323, -299.1323897829857970, -207.2190165580626910 ) ) ;
#28441=CARTESIAN_POINT ( 'NONE',  ( 10.44029577962546185, -282.1220172704596507, -210.6654071994988726 ) ) ;
#28442=CARTESIAN_POINT ( 'NONE',  ( -109.6445023313047216, -294.2996289942353201, -291.6366537529475522 ) ) ;
#28443=CARTESIAN_POINT ( 'NONE',  ( 33.45558131864618190, -281.3166696193655412, -252.5130019504298104 ) ) ;
#28444=CARTESIAN_POINT ( 'NONE',  ( -92.69552985178474103, -295.9855633861066053, -323.8863787425185023 ) ) ;
#28445=CARTESIAN_POINT ( 'NONE',  ( -55.48289355846002024, -299.3347238296130399, -198.8827869876849377 ) ) ;
#28446=CARTESIAN_POINT ( 'NONE',  ( 21.87882984116004437, -284.9918841294445429, -223.4124239601724469 ) ) ;
#28447=CARTESIAN_POINT ( 'NONE',  ( -31.26196546129850873, -282.1289783527839177, -195.5566186812525586 ) ) ;
#28448=CARTESIAN_POINT ( 'NONE',  ( -84.21627007210248905, -296.4480018408657429, -214.0260687512058837 ) ) ;
#28450=CYLINDRICAL_SURFACE ( 'NONE', #74062, 2.397123461337413719 ) ;
#28451=CARTESIAN_POINT ( 'NONE',  ( 4.328879329303341628, -284.4675369076890661, -332.3543386368593247 ) ) ;
#28453=CARTESIAN_POINT ( 'NONE',  ( -37.37352853689063181, -292.5523547857347353, -345.3611179825600175 ) ) ;
#28454=CARTESIAN_POINT ( 'NONE',  ( 37.13125224652835499, -274.5120875601161856, -251.4418636189326719 ) ) ;
#28455=CARTESIAN_POINT ( 'NONE',  ( -1.254829195941062903, -292.3784751178791907, -206.8900608952109224 ) ) ;
#28456=CARTESIAN_POINT ( 'NONE',  ( 21.57577524728873897, -283.6882023982014402, -314.6475266157881947 ) ) ;
#28457=CARTESIAN_POINT ( 'NONE',  ( 27.32783823085941677, -276.6705761294236368, -234.6977897020352941 ) ) ;
#28458=CARTESIAN_POINT ( 'NONE',  ( -33.08287447289618655, -284.5995056645817840, -346.4550129270340335 ) ) ;
#28459=CARTESIAN_POINT ( 'NONE',  ( 30.39380530294350891, -279.9699497601903317, -242.0939672980213970 ) ) ;
#28460=CARTESIAN_POINT ( 'NONE',  ( -112.3932127978049209, -280.5483375756771807, -270.6710630290847917 ) ) ;
#28461=CARTESIAN_POINT ( 'NONE',  ( -48.96998934205065979, -297.9080622941874594, -194.1905487919816835 ) ) ;
#28462=CARTESIAN_POINT ( 'NONE',  ( 32.55395254745287303, -274.9707405430401082, -237.9293751423893752 ) ) ;
#28463=CARTESIAN_POINT ( 'NONE',  ( 17.78850000220721483, -294.7687040044921787, -220.2657980348386104 ) ) ;
#28465=EDGE_CURVE ( 'NONE', #71834, #82501, #31333, .T. ) ;
#28467=CARTESIAN_POINT ( 'NONE',  ( -25.13061993587638909, -293.0377698050264144, -345.1886075569556169 ) ) ;
#28469=CARTESIAN_POINT ( 'NONE',  ( -90.23683606011185532, -272.7861916843015706, -219.9434803805021375 ) ) ;
#28470=CARTESIAN_POINT ( 'NONE',  ( -8.630782098019755821, -296.2034329184634771, -341.1163975170875347 ) ) ;
#28471=CARTESIAN_POINT ( 'NONE',  ( 21.89240877794877704, -294.1015500400542351, -221.7881927840422236 ) ) ;
#28472=CARTESIAN_POINT ( 'NONE',  ( -31.70854943656532043, -290.9811823333152461, -345.0340290010827289 ) ) ;
#28473=CARTESIAN_POINT ( 'NONE',  ( -110.5637862384032530, -276.3532372914447137, -285.8063287626636111 ) ) ;
#28474=CARTESIAN_POINT ( 'NONE',  ( -69.85879053232243052, -279.4038289387650593, -337.3375516678631811 ) ) ;
#28475=CARTESIAN_POINT ( 'NONE',  ( 27.02579904642238517, -292.1350876887759682, -307.7528182094750377 ) ) ;
#28476=CARTESIAN_POINT ( 'NONE',  ( 24.11939543188977453, -284.0097929729437283, -314.6870908671187976 ) ) ;
#28477=CARTESIAN_POINT ( 'NONE',  ( -60.06143061898620772, -284.6709599091000769, -200.6614772407775149 ) ) ;
#28479=CARTESIAN_POINT ( 'NONE',  ( -69.02217679628078884, -283.1473695424714947, -336.1657673458254294 ) ) ;
#28480=CARTESIAN_POINT ( 'NONE',  ( 19.88881048564466170, -281.9366943835040615, -219.2908015978099741 ) ) ;
#28481=CARTESIAN_POINT ( 'NONE',  ( -75.89354559437660441, -284.3446289529159117, -204.1051473292179423 ) ) ;
#28482=CARTESIAN_POINT ( 'NONE',  ( -99.24525265291504184, -280.0983648947290021, -224.9432197278113676 ) ) ;
#28484=CARTESIAN_POINT ( 'NONE',  ( -42.73764658997463783, -278.6391963444464182, -346.4767636455488287 ) ) ;
#28485=CARTESIAN_POINT ( 'NONE',  ( -107.3417001280813565, -270.0523547857346784, -270.3292895737509980 ) ) ;
#28488=CARTESIAN_POINT ( 'NONE',  ( 98.92740146068138074, -301.7582495827366529, -195.3146565631489864 ) ) ;
#28489=CARTESIAN_POINT ( 'NONE',  ( -52.12907782588145267, -277.8821703048455447, -197.1427941626550933 ) ) ;
#28490=CARTESIAN_POINT ( 'NONE',  ( -109.8085733308718375, -292.0192256045564250, -293.3916848779560382 ) ) ;
#28491=CARTESIAN_POINT ( 'NONE',  ( 33.21290587866195665, -293.1536491949343599, -289.5382562690976442 ) ) ;
#28492=CARTESIAN_POINT ( 'NONE',  ( -37.50775581640981926, -288.5617982835651105, -347.3124618552888023 ) ) ;
#28494=CARTESIAN_POINT ( 'NONE',  ( 35.80033258094827886, -292.4085891141127149, -292.6501493059306540 ) ) ;
#28495=CARTESIAN_POINT ( 'NONE',  ( 13.70748821460256650, -285.1814993094901638, -216.9949957669825551 ) ) ;
#28496=CARTESIAN_POINT ( 'NONE',  ( -52.64719312274739593, -293.7145564622181837, -197.6680753076331882 ) ) ;
#28497=CARTESIAN_POINT ( 'NONE',  ( -30.44732214321059516, -284.6206489963906279, -196.9397109779411608 ) ) ;
#28498=CARTESIAN_POINT ( 'NONE',  ( 33.43888422345286671, -283.1270411310507598, -290.1437456567363142 ) ) ;
#28499=CARTESIAN_POINT ( 'NONE',  ( -16.70143513112662959, -293.2537280737448668, -196.4233084857097822 ) ) ;
#28500=CARTESIAN_POINT ( 'NONE',  ( 32.79190502860596723, -281.7738542076801878, -249.8851352351114485 ) ) ;
#28501=CARTESIAN_POINT ( 'NONE',  ( -36.29534569271209676, -293.8342745126162754, -346.9699366343728570 ) ) ;
#28502=CARTESIAN_POINT ( 'NONE',  ( -43.15984973873052866, -289.9266858464213215, -346.9790529299918376 ) ) ;
#28503=CARTESIAN_POINT ( 'NONE',  ( -26.14731371219676603, -289.4056175643074198, -346.4808435198353891 ) ) ;
#28504=CARTESIAN_POINT ( 'NONE',  ( -89.66433739983241935, -285.4556235800654349, -219.3833542634595517 ) ) ;
#28507=CARTESIAN_POINT ( 'NONE',  ( -41.84802413041015967, -296.9686393303921932, -346.0433434733269564 ) ) ;
#28508=CARTESIAN_POINT ( 'NONE',  ( -50.39993521719393499, -293.9002168524291392, -345.7989399140182059 ) ) ;
#28509=CARTESIAN_POINT ( 'NONE',  ( -110.5157259006389268, -277.5715116476278013, -273.3561805335664872 ) ) ;
#28510=CARTESIAN_POINT ( 'NONE',  ( -60.84635035476559040, -273.2628992908906298, -197.0453243812449102 ) ) ;
#28511=CARTESIAN_POINT ( 'NONE',  ( 12.81270761395191826, -292.8172340018795126, -324.4240326373146672 ) ) ;
#28512=CARTESIAN_POINT ( 'NONE',  ( 18.21044641385283569, -278.0012426477495069, -319.2876373444584601 ) ) ;
#28513=CARTESIAN_POINT ( 'NONE',  ( -111.5769001271280843, -270.6920356235430631, -270.3374848783465154 ) ) ;
#28514=CARTESIAN_POINT ( 'NONE',  ( 18.28334148698370143, -295.4356552216946739, -318.2654117656361450 ) ) ;
#28515=CARTESIAN_POINT ( 'NONE',  ( -84.66721260088756651, -296.8016400516380600, -326.4145592287690079 ) ) ;
#28517=CARTESIAN_POINT ( 'NONE',  ( -87.40385372127317964, -293.7478560322562657, -326.5006183914676967 ) ) ;
#28518=CARTESIAN_POINT ( 'NONE',  ( -60.12581276806698583, -298.4159258269825159, -196.8604699823577562 ) ) ;
#28519=CARTESIAN_POINT ( 'NONE',  ( -56.23423490102257460, -287.8749300005506484, -341.5368630525657068 ) ) ;
#28520=CARTESIAN_POINT ( 'NONE',  ( -96.19763085118555068, -275.1907627763315531, -223.8747751254295508 ) ) ;
#28521=CARTESIAN_POINT ( 'NONE',  ( -109.9349923283016324, -291.6255911271211403, -260.3086581466929488 ) ) ;
#28522=CARTESIAN_POINT ( 'NONE',  ( -34.11205789542941602, -274.5840959186526788, -193.4904713453673253 ) ) ;
#28523=CARTESIAN_POINT ( 'NONE',  ( -108.6115791286629815, -296.6757965447201855, -286.2574016400802179 ) ) ;
#28524=CARTESIAN_POINT ( 'NONE',  ( -102.0132352982649309, -281.0485310563680628, -231.5814530067391956 ) ) ;
#28525=CARTESIAN_POINT ( 'NONE',  ( 37.20083460002793885, -280.0195157330298912, -253.0782653648941505 ) ) ;
#28526=EDGE_LOOP ( 'NONE', ( #79054, #15330 ) ) ;
#28528=CARTESIAN_POINT ( 'NONE',  ( -69.15187290582098001, -282.8082658700704428, -340.3856966308424603 ) ) ;
#28529=CARTESIAN_POINT ( 'NONE',  ( 26.85004453705635896, -274.3432348589163894, -228.0204436447908449 ) ) ;
#28530=CARTESIAN_POINT ( 'NONE',  ( -25.49961332998155328, -278.6005328050862317, -195.0869165981462459 ) ) ;
#28531=CARTESIAN_POINT ( 'NONE',  ( 18.77732092554002463, -278.8573599125859914, -220.3349179597435636 ) ) ;
#28533=CARTESIAN_POINT ( 'NONE',  ( -95.06368389007577946, -271.7658846459888764, -224.7152253996716524 ) ) ;
#28534=CARTESIAN_POINT ( 'NONE',  ( 11.83664892150792447, -276.7349936858275896, -213.6674257877280638 ) ) ;
#28537=CARTESIAN_POINT ( 'NONE',  ( 32.93814406427365782, -291.2186798921856052, -243.0294737510616301 ) ) ;
#28538=CARTESIAN_POINT ( 'NONE',  ( -107.2604300942438584, -290.9661963431117329, -237.9792970038828344 ) ) ;
#28539=CARTESIAN_POINT ( 'NONE',  ( 28.93879108266040134, -278.0229503649280787, -305.9242239625236834 ) ) ;
#28540=CARTESIAN_POINT ( 'NONE',  ( -90.64620244883043654, -271.2964016184525349, -217.6009940230856898 ) ) ;
#28541=CARTESIAN_POINT ( 'NONE',  ( -65.80801644476309775, -284.8863002828427398, -198.9759378816672779 ) ) ;
#28543=CARTESIAN_POINT ( 'NONE',  ( -110.4605518797364567, -282.7670474610935685, -253.6123716280919211 ) ) ;
#28545=CARTESIAN_POINT ( 'NONE',  ( 34.60876271578055707, -292.1568240332521782, -255.8607247996800709 ) ) ;
#28546=CARTESIAN_POINT ( 'NONE',  ( 28.76876495960400248, -285.2392658908804606, -236.4797965107975983 ) ) ;
#28549=CARTESIAN_POINT ( 'NONE',  ( 0.2222790942726419194, -292.5521961339405266, -335.3353120175667073 ) ) ;
#28550=CARTESIAN_POINT ( 'NONE',  ( -71.44638962548887662, -281.9742861700697745, -338.6222189808248686 ) ) ;
#28551=CARTESIAN_POINT ( 'NONE',  ( -71.32802330024252058, -281.1957769393596891, -204.8383234104281314 ) ) ;
#28552=CARTESIAN_POINT ( 'NONE',  ( -112.7433490751408840, -285.5836919336028927, -284.1649993788072379 ) ) ;
#28553=CARTESIAN_POINT ( 'NONE',  ( -4.080656119599637144, -278.7245511021169477, -202.0263889879495878 ) ) ;
#28554=CARTESIAN_POINT ( 'NONE',  ( 32.31361609759608911, -287.8436563150969505, -292.3728220202745547 ) ) ;
#28555=CARTESIAN_POINT ( 'NONE',  ( -93.16183596830248348, -279.3001362223347428, -318.3140882050001323 ) ) ;
#28556=CARTESIAN_POINT ( 'NONE',  ( -76.43347931896123271, -278.3921269405136627, -332.2627079808701183 ) ) ;
#28557=CARTESIAN_POINT ( 'NONE',  ( -108.4340450161021181, -286.8541073822441376, -245.3754160728247484 ) ) ;
#28559=CARTESIAN_POINT ( 'NONE',  ( -78.20066584281454425, -297.3520132355545798, -205.0959287526150945 ) ) ;
#28560=CARTESIAN_POINT ( 'NONE',  ( -26.20514170116859987, -290.8897307150051006, -344.2226944491937957 ) ) ;
#28562=CARTESIAN_POINT ( 'NONE',  ( -55.63300648810263738, -288.3376638359845288, -190.3683826091709363 ) ) ;
#28564=CARTESIAN_POINT ( 'NONE',  ( -43.85782345427671203, -271.9699448503430972, -195.4253793298688890 ) ) ;
#28565=CARTESIAN_POINT ( 'NONE',  ( 31.49845563045568397, -292.3765361795876174, -303.1562621562962931 ) ) ;
#28566=CARTESIAN_POINT ( 'NONE',  ( -40.01830389208569017, -287.5380362941845078, -196.7164063859355565 ) ) ;
#28568=CARTESIAN_POINT ( 'NONE',  ( 36.35922337219032130, -283.2169009494947431, -263.0289747195490691 ) ) ;
#28569=CARTESIAN_POINT ( 'NONE',  ( -23.40148035319239739, -290.3026962991718278, -345.5432208753875329 ) ) ;
#28570=CARTESIAN_POINT ( 'NONE',  ( -15.07963746813612360, -290.0850202617360765, -343.6128194289748876 ) ) ;
#28571=CARTESIAN_POINT ( 'NONE',  ( -40.28811120983795746, -285.0893599131707674, -345.3032243909405565 ) ) ;
#28572=CARTESIAN_POINT ( 'NONE',  ( -62.40398497116377996, -277.5359233304245095, -343.2245811122954251 ) ) ;
#28574=CARTESIAN_POINT ( 'NONE',  ( 32.08363315579531871, -292.0206311653488456, -300.3165891057225849 ) ) ;
#28575=CARTESIAN_POINT ( 'NONE',  ( 37.54787317587523177, -281.6100430444549829, -288.3213134733172183 ) ) ;
#28576=CARTESIAN_POINT ( 'NONE',  ( -38.11866273645279790, -275.9027303578936312, -196.1299802249641857 ) ) ;
#28577=CARTESIAN_POINT ( 'NONE',  ( -37.30987171927208124, -285.5519495502701943, -345.3611179825600175 ) ) ;
#28578=CARTESIAN_POINT ( 'NONE',  ( 38.31072428392599249, -273.6949852128341831, -262.7050263693009811 ) ) ;
#28580=CARTESIAN_POINT ( 'NONE',  ( -35.65509781019719071, -279.5814970969258866, -197.3066360357894666 ) ) ;
#28581=CARTESIAN_POINT ( 'NONE',  ( 37.79590505368462061, -276.9446766378411553, -285.2724897271040163 ) ) ;
#28582=CARTESIAN_POINT ( 'NONE',  ( -41.92301125775718873, -299.4185651724802142, -196.9146306187143125 ) ) ;
#28583=CARTESIAN_POINT ( 'NONE',  ( -83.75051943416367806, -282.7301404120939310, -331.5756036024696982 ) ) ;
#28584=CARTESIAN_POINT ( 'NONE',  ( -107.9753013925963501, -292.6018137217848789, -248.2080133815861984 ) ) ;
#28585=CARTESIAN_POINT ( 'NONE',  ( -21.54077395617752799, -275.8516179978487912, -195.8173647531914412 ) ) ;
#28587=CARTESIAN_POINT ( 'NONE',  ( 98.29621670120258159, -300.9199634798632133, -193.7310287357714742 ) ) ;
#28589=CARTESIAN_POINT ( 'NONE',  ( -35.58260892391334806, -297.0302193835679532, -345.1865871620890971 ) ) ;
#28590=CARTESIAN_POINT ( 'NONE',  ( -26.50176542822750037, -280.9138818148171595, -344.4577733266178825 ) ) ;
#28591=CARTESIAN_POINT ( 'NONE',  ( -111.9026155549361476, -289.9786608994671724, -289.5558101779715230 ) ) ;
#28592=CARTESIAN_POINT ( 'NONE',  ( 33.65498902118835645, -273.8713452967687658, -293.4114310478694847 ) ) ;
#28593=CARTESIAN_POINT ( 'NONE',  ( 29.42071459036348102, -288.6703062843075145, -233.5199520612079596 ) ) ;
#28594=CARTESIAN_POINT ( 'NONE',  ( -101.9219384145607989, -289.0001049265405300, -305.1619944745023645 ) ) ;
#28596=CARTESIAN_POINT ( 'NONE',  ( -96.84277371914417643, -288.4790977218034982, -318.3216007486200851 ) ) ;
#28597=CARTESIAN_POINT ( 'NONE',  ( -95.78779648069846075, -289.6043659490258051, -314.1557378135203180 ) ) ;
#28598=ORIENTED_EDGE ( 'NONE', *, *, #61048, .F. ) ;
#28599=CARTESIAN_POINT ( 'NONE',  ( -54.90721545993856978, -286.9110891317310461, -195.7089567278675020 ) ) ;
#28600=CARTESIAN_POINT ( 'NONE',  ( -66.80730314165892025, -277.7825002068363460, -337.1732854813812423 ) ) ;
#28601=CARTESIAN_POINT ( 'NONE',  ( 29.29922972513464785, -292.9685751236604005, -308.4220048040718893 ) ) ;
#28602=CARTESIAN_POINT ( 'NONE',  ( -109.2047295540654943, -284.8549974712008748, -297.8776432634088565 ) ) ;
#28603=CARTESIAN_POINT ( 'NONE',  ( -67.18478086484179812, -286.0047023192887536, -199.4024340622470390 ) ) ;
#28605=CARTESIAN_POINT ( 'NONE',  ( -35.66656833962258588, -280.4069919106366342, -197.3467840251825862 ) ) ;
#28606=CARTESIAN_POINT ( 'NONE',  ( 199.9431822037543895, 289.4637811216681484, -97.53612682803708367 ) ) ;
#28607=CARTESIAN_POINT ( 'NONE',  ( 172.7456591032144217, 243.4255081464518469, -179.1439596359693951 ) ) ;
#28608=CARTESIAN_POINT ( 'NONE',  ( 199.8454374018455155, 291.1247744847867693, -82.44697178725743925 ) ) ;
#28609=CARTESIAN_POINT ( 'NONE',  ( -105.5631175224678060, -272.1033404182197160, -243.7934079629947348 ) ) ;
#28610=CARTESIAN_POINT ( 'NONE',  ( 11.76373686284951248, -273.6732817008837060, -215.8603904072934085 ) ) ;
#28611=CARTESIAN_POINT ( 'NONE',  ( -93.64871248334942777, -295.3443503549772799, -322.8118811401897688 ) ) ;
#28612=CARTESIAN_POINT ( 'NONE',  ( 197.3573331818941199, 281.6218204230049764, -110.3645358861669621 ) ) ;
#28613=CARTESIAN_POINT ( 'NONE',  ( -89.81238187975995402, -272.0152907662348412, -214.6100140034042738 ) ) ;
#28614=CARTESIAN_POINT ( 'NONE',  ( -82.71754104506084104, -299.2852353268698948, -211.5430932386634311 ) ) ;
#28615=CARTESIAN_POINT ( 'NONE',  ( -26.38493765066929697, -290.2251195794141267, -343.0843292747882742 ) ) ;
#28616=CARTESIAN_POINT ( 'NONE',  ( -47.04894798124955457, -293.0056245913336852, -197.6975410527181225 ) ) ;
#28618=CARTESIAN_POINT ( 'NONE',  ( -112.6601639414535896, -297.6802952042838797, -255.4627805770078908 ) ) ;
#28619=CARTESIAN_POINT ( 'NONE',  ( -62.59001911922237582, -286.2070151452742834, -201.7468910568526894 ) ) ;
#28620=CARTESIAN_POINT ( 'NONE',  ( 27.97406667447834749, -294.8865092217719734, -310.9334298753838652 ) ) ;
#28621=CARTESIAN_POINT ( 'NONE',  ( 1.743578206831889688, -295.0363330136170248, -336.6322875867046491 ) ) ;
#28622=CARTESIAN_POINT ( 'NONE',  ( 20.18158153086591611, -293.0850774663261404, -225.3956698767600528 ) ) ;
#28624=CARTESIAN_POINT ( 'NONE',  ( -66.99350518999349902, -275.5866846015036344, -200.8623075148435646 ) ) ;
#28626=CARTESIAN_POINT ( 'NONE',  ( -69.93060055712770406, -279.1420517671097059, -200.6510414866850738 ) ) ;
#28627=PRODUCT_DEFINITION_CONTEXT ( 'detailed design', #62598, 'design' ) ;
#28628=CARTESIAN_POINT ( 'NONE',  ( 35.16323437238900596, -273.7724060376565376, -256.5961301584999319 ) ) ;
#28629=CARTESIAN_POINT ( 'NONE',  ( -35.14814744777818589, -299.2852899822167956, -196.9635804436839521 ) ) ;
#28630=CARTESIAN_POINT ( 'NONE',  ( 11.69520675621157579, -275.6938797878317473, -215.8980822190610809 ) ) ;
#28631=CARTESIAN_POINT ( 'NONE',  ( -57.86969819946626359, -275.5508479452520874, -197.1451213531220787 ) ) ;
#28632=CARTESIAN_POINT ( 'NONE',  ( 36.03911415418804154, -273.3526174624257123, -253.1683092593688968 ) ) ;
#28633=CARTESIAN_POINT ( 'NONE',  ( -108.0660898847512925, -296.9591701710171492, -288.9025687809136684 ) ) ;
#28634=CARTESIAN_POINT ( 'NONE',  ( 30.02221297379228560, -292.5222135302249740, -299.9833752756852050 ) ) ;
#28636=CARTESIAN_POINT ( 'NONE',  ( -114.1702220533711341, -278.9930361417931977, -274.4727018439157291 ) ) ;
#28637=CARTESIAN_POINT ( 'NONE',  ( 20.02377983392060656, -276.3558815742215984, -315.5276970628954700 ) ) ;
#28638=CARTESIAN_POINT ( 'NONE',  ( -54.83547755593648532, -284.5166291460943739, -195.8811473681408017 ) ) ;
#28639=CARTESIAN_POINT ( 'NONE',  ( -15.50192490817703472, -300.3250948112315655, -195.1870173997247377 ) ) ;
#28641=CARTESIAN_POINT ( 'NONE',  ( 27.16803260128937580, -287.2200307440771212, -304.9811733557868934 ) ) ;
#28642=CARTESIAN_POINT ( 'NONE',  ( -102.7629399610539451, -276.3270049458675430, -304.9737658125844177 ) ) ;
#28643=CARTESIAN_POINT ( 'NONE',  ( -96.07111906590684214, -277.7450392750235437, -225.9980127734212090 ) ) ;
#28644=CARTESIAN_POINT ( 'NONE',  ( -112.3926082005458085, -286.5555504912839524, -270.1093041087452775 ) ) ;
#28645=CARTESIAN_POINT ( 'NONE',  ( -56.69014825028757798, -278.5121529209635582, -341.2148023865774462 ) ) ;
#28647=CARTESIAN_POINT ( 'NONE',  ( 37.39372394057577509, -274.1399261341155125, -285.2290972235209097 ) ) ;
#28648=CARTESIAN_POINT ( 'NONE',  ( 30.26593218869695789, -275.8298379601324655, -242.4235477907718632 ) ) ;
#28649=CARTESIAN_POINT ( 'NONE',  ( 25.21069362367574840, -284.1142764797457971, -312.0411667167350060 ) ) ;
#28651=CARTESIAN_POINT ( 'NONE',  ( 36.31039383494378825, -289.2566057811712881, -253.4312189103996502 ) ) ;
#28652=CARTESIAN_POINT ( 'NONE',  ( 17.42841982436524972, -292.2700949125618308, -321.6728848860828407 ) ) ;
#28653=ADVANCED_FACE ( 'NONE', ( #8606, #45499 ), #16189, .T. ) ;
#28655=CARTESIAN_POINT ( 'NONE',  ( -19.13335423497906262, -272.9761024779716081, -199.1065105522791896 ) ) ;
#28656=CARTESIAN_POINT ( 'NONE',  ( 2.930151069906376193, -290.7381477128460574, -207.9380173828699299 ) ) ;
#28657=CARTESIAN_POINT ( 'NONE',  ( -28.16072294498304274, -126.4832272301380556, -368.1402060870429409 ) ) ;
#28659=CARTESIAN_POINT ( 'NONE',  ( -36.11755601511399050, -287.5169839217354593, -346.6709599171697960 ) ) ;
#28660=CARTESIAN_POINT ( 'NONE',  ( -87.45731342431548683, -285.3651013704769639, -324.6054151949148263 ) ) ;
#28661=CARTESIAN_POINT ( 'NONE',  ( -111.3674071488271409, -283.0093818693535468, -253.2097705752599097 ) ) ;
#28662=CARTESIAN_POINT ( 'NONE',  ( -8.244693324677454527, -284.0887481021479175, -337.9535666237158011 ) ) ;
#28663=CARTESIAN_POINT ( 'NONE',  ( -108.5249953298580436, -285.5780629189009687, -253.4091958844059036 ) ) ;
#28664=CARTESIAN_POINT ( 'NONE',  ( -98.70659666386923448, -293.1239175678067568, -226.6260487877287346 ) ) ;
#28666=CARTESIAN_POINT ( 'NONE',  ( -92.15698610461994633, -273.6279996527131289, -216.3145758656163196 ) ) ;
#28667=CARTESIAN_POINT ( 'NONE',  ( -110.1608738582254290, -288.3745377523694060, -290.5274795062143198 ) ) ;
#28668=CARTESIAN_POINT ( 'NONE',  ( -3.994849273332384598, -276.6244627062955033, -339.7801377912581415 ) ) ;
#28670=CARTESIAN_POINT ( 'NONE',  ( 37.26449636698217205, -295.5010816555038105, -267.9606504731878545 ) ) ;
#28672=CARTESIAN_POINT ( 'NONE',  ( -54.42813229853333468, -297.7662352645559167, -345.3683826091709648 ) ) ;
#28673=CARTESIAN_POINT ( 'NONE',  ( -90.00462221785272732, -283.9740084339952659, -219.0254483009370858 ) ) ;
#28674=CARTESIAN_POINT ( 'NONE',  ( -89.64468680142144308, -277.3149834520348804, -216.5356183031331057 ) ) ;
#28675=CARTESIAN_POINT ( 'NONE',  ( -55.15283607664092358, -272.3069708041207946, -196.1622555444353964 ) ) ;
#28677=CARTESIAN_POINT ( 'NONE',  ( 35.45476189744334050, -274.9886787818614948, -277.0370287497797221 ) ) ;
#28678=CARTESIAN_POINT ( 'NONE',  ( 15.35791437019653038, -294.3332629596289962, -218.7763194314568409 ) ) ;
#28679=CARTESIAN_POINT ( 'NONE',  ( 26.00216572862364117, -294.9960329119103903, -307.1165679997777715 ) ) ;
#28680=CARTESIAN_POINT ( 'NONE',  ( -74.35301600703208180, -296.8484562379771319, -337.3790920864740883 ) ) ;
#28681=CARTESIAN_POINT ( 'NONE',  ( -106.7061191744315352, -296.6893236095895077, -247.4505508893097954 ) ) ;
#28682=CARTESIAN_POINT ( 'NONE',  ( -74.51469973401995617, -291.5467401008506840, -335.5155315235590479 ) ) ;
#28683=CARTESIAN_POINT ( 'NONE',  ( -66.57428434567681563, -283.5912626331861475, -341.6105198614217215 ) ) ;
#28684=CARTESIAN_POINT ( 'NONE',  ( -21.58812544718778170, -272.3916306235416869, -196.2522091890145930 ) ) ;
#28685=CARTESIAN_POINT ( 'NONE',  ( 22.09152783232254436, -286.7277218172623066, -221.4051028389808664 ) ) ;
#28686=CARTESIAN_POINT ( 'NONE',  ( -10.64269782588093172, -278.6820632574600722, -340.0677179490696744 ) ) ;
#28687=CARTESIAN_POINT ( 'NONE',  ( -97.54254689361944486, -284.1903460932551297, -228.6344419062922668 ) ) ;
#28688=CARTESIAN_POINT ( 'NONE',  ( -45.82551048213237976, -287.1594166383063111, -344.9314914214473902 ) ) ;
#28689=CARTESIAN_POINT ( 'NONE',  ( 133.9787772367566561, 181.9811788097603937, -239.6702418147338562 ) ) ;
#28690=CARTESIAN_POINT ( 'NONE',  ( -46.72656677273066350, -285.4375796011000830, -197.8540185774890574 ) ) ;
#28691=CARTESIAN_POINT ( 'NONE',  ( 36.21412361271706715, -282.4870526845435279, -248.9237189662935350 ) ) ;
#28692=CARTESIAN_POINT ( 'NONE',  ( -37.51313324917455105, -288.1129661712404300, -347.1386650677256966 ) ) ;
#28693=CARTESIAN_POINT ( 'NONE',  ( -64.47670133170277040, -281.3040613688663143, -199.1006054706350028 ) ) ;
#28695=CARTESIAN_POINT ( 'NONE',  ( -101.6731843001405338, -279.3193833865271358, -311.8673988259027965 ) ) ;
#28696=CARTESIAN_POINT ( 'NONE',  ( -99.46661477659858974, -278.9152176534990417, -231.9306962631322051 ) ) ;
#28697=CARTESIAN_POINT ( 'NONE',  ( -88.47805353815522267, -275.3113733633115316, -215.9127545520194644 ) ) ;
#28698=CARTESIAN_POINT ( 'NONE',  ( 39.71162069869933475, -293.5515123490475276, -270.3099585778629148 ) ) ;
#28699=CARTESIAN_POINT ( 'NONE',  ( 24.08952345884162227, -286.1500996849189846, -312.7870759143351620 ) ) ;
#28700=CARTESIAN_POINT ( 'NONE',  ( -37.81076760605006370, -293.6464904254155499, -194.1625589780649079 ) ) ;
#28701=CARTESIAN_POINT ( 'NONE',  ( -109.5781130771610918, -295.6366126532654448, -257.8660502213547261 ) ) ;
#28702=CARTESIAN_POINT ( 'NONE',  ( 35.90670947416063541, -283.6448476284422782, -283.6985933199347301 ) ) ;
#28703=CARTESIAN_POINT ( 'NONE',  ( -108.4966853032510130, -296.4351901858185556, -253.9582044729913264 ) ) ;
#28704=CARTESIAN_POINT ( 'NONE',  ( -33.56838050155253939, -293.1782717564379936, -193.7631116818319299 ) ) ;
#28705=CARTESIAN_POINT ( 'NONE',  ( -16.90115065487985646, -280.9746345604610838, -200.1751036696183803 ) ) ;
#28706=CARTESIAN_POINT ( 'NONE',  ( 13.81662648194687470, -273.8073065629759526, -213.0568152703448277 ) ) ;
#28707=CARTESIAN_POINT ( 'NONE',  ( -62.72217063166173290, -290.0252844656328080, -343.0062984609721752 ) ) ;
#28708=CARTESIAN_POINT ( 'NONE',  ( -64.82654988485565184, -281.5468771600368427, -340.9788388213065105 ) ) ;
#28709=CARTESIAN_POINT ( 'NONE',  ( -112.6201884736154852, -291.0874582914054827, -254.2087439842300398 ) ) ;
#28710=CARTESIAN_POINT ( 'NONE',  ( -23.77708614465076664, -289.2074546971101654, -342.1630151821632353 ) ) ;
#28712=CARTESIAN_POINT ( 'NONE',  ( 119.9254157080543877, 149.4800609170424366, -261.9094989083125142 ) ) ;
#28713=CARTESIAN_POINT ( 'NONE',  ( 6.105808943458286286, -59.49341857825391600, -350.9694942175905226 ) ) ;
#28714=CARTESIAN_POINT ( 'NONE',  ( -37.30987171927208834, -277.5523547857346784, -195.3611179825600175 ) ) ;
#28715=CARTESIAN_POINT ( 'NONE',  ( -74.57918986198156119, -278.7405550429625123, -207.3269355501208508 ) ) ;
#28717=CARTESIAN_POINT ( 'NONE',  ( -85.67772412041780683, -278.2846146422053835, -215.2443795324813038 ) ) ;
#28718=CARTESIAN_POINT ( 'NONE',  ( -2.563298046150888521, -274.1661232291770034, -201.6717726205803558 ) ) ;
#28719=CARTESIAN_POINT ( 'NONE',  ( 169.1947799176787726, 229.7990775681149671, -190.7372803930986436 ) ) ;
#28720=CARTESIAN_POINT ( 'NONE',  ( -70.95888190455409017, -278.1919750086883596, -201.7426701361403332 ) ) ;
#28721=CARTESIAN_POINT ( 'NONE',  ( -81.62167398621286907, -281.6778557905246885, -330.5181259571628516 ) ) ;
#28722=CARTESIAN_POINT ( 'NONE',  ( -88.93691533465818111, -299.0995654029789534, -214.5053440036580525 ) ) ;
#28723=CARTESIAN_POINT ( 'NONE',  ( -90.80849229721653160, -291.7600144409868790, -220.5501434730140602 ) ) ;
#28724=CARTESIAN_POINT ( 'NONE',  ( 18.18720715152066703, -286.9191921688429261, -318.5806597389935746 ) ) ;
#28725=CARTESIAN_POINT ( 'NONE',  ( -55.31784767184479534, -274.4781564887141485, -195.5936724881837847 ) ) ;
#28726=CARTESIAN_POINT ( 'NONE',  ( -105.4162409253727191, -272.9060437272266313, -243.8615407598908575 ) ) ;
#28730=CARTESIAN_POINT ( 'NONE',  ( -90.07111969060639467, -281.2346664249291166, -216.1686317819166732 ) ) ;
#28733=CARTESIAN_POINT ( 'NONE',  ( 13.53979385763831722, -281.8644239470314119, -217.5144513001816904 ) ) ;
#28734=CARTESIAN_POINT ( 'NONE',  ( -70.80875313821908890, -281.3768728751016965, -202.1413966379129761 ) ) ;
#28736=CARTESIAN_POINT ( 'NONE',  ( -110.4623556885065767, -283.6756369416274310, -265.4374810263855125 ) ) ;
#28737=CARTESIAN_POINT ( 'NONE',  ( -109.0066130346584146, -280.1610287093493525, -289.7261829295458142 ) ) ;
#28738=CARTESIAN_POINT ( 'NONE',  ( -24.45635332049452870, -272.6993305283129985, -197.7509529244380531 ) ) ;
#28741=CARTESIAN_POINT ( 'NONE',  ( -25.78414542985145275, -277.7113298125578353, -346.3254632341079287 ) ) ;
#28743=CARTESIAN_POINT ( 'NONE',  ( -107.0460999122108348, -276.7225593208636383, -301.7933369777632038 ) ) ;
#28746=CARTESIAN_POINT ( 'NONE',  ( -78.24530373153159246, -285.5793213021553356, -333.6485734020911309 ) ) ;
#28747=CARTESIAN_POINT ( 'NONE',  ( 18.60666309637325710, -292.0810507775216820, -223.2189672050852209 ) ) ;
#28748=CARTESIAN_POINT ( 'NONE',  ( -5.676057623411916886, -287.9951255879259975, -340.4367904498428175 ) ) ;
#28749=CARTESIAN_POINT ( 'NONE',  ( -65.45768030036708751, -283.9194548355274037, -201.8415027783975972 ) ) ;
#28750=CARTESIAN_POINT ( 'NONE',  ( -108.5946758337290277, -283.3677698945090810, -251.9657823873016014 ) ) ;
#28751=CARTESIAN_POINT ( 'NONE',  ( 20.28859750513982974, -286.4396493854808909, -316.8016478173460087 ) ) ;
#28752=CARTESIAN_POINT ( 'NONE',  ( 16.12559053676564957, -283.4778493002770574, -320.7174535654094143 ) ) ;
#28753=CARTESIAN_POINT ( 'NONE',  ( -54.84159006591922036, -271.8270095311204386, -197.4313264169590525 ) ) ;
#28754=CARTESIAN_POINT ( 'NONE',  ( -102.2474340195895337, -282.4248041733705463, -310.2821164963623346 ) ) ;
#28755=CARTESIAN_POINT ( 'NONE',  ( -69.91558977714404932, -297.4812203197503209, -337.9322058239084186 ) ) ;
#28756=CARTESIAN_POINT ( 'NONE',  ( -29.62520417999557765, -284.1495032152307090, -195.5915779538694892 ) ) ;
#28757=CARTESIAN_POINT ( 'NONE',  ( -72.25239122059259955, -280.5194574870578776, -205.9821455148923519 ) ) ;
#28758=CARTESIAN_POINT ( 'NONE',  ( 6.454555433670044806, -288.6453714791052789, -209.2076132912932849 ) ) ;
#28761=CARTESIAN_POINT ( 'NONE',  ( 18.33769170834741757, -294.7640749977289829, -219.2815768396147860 ) ) ;
#28762=CARTESIAN_POINT ( 'NONE',  ( -79.78422865670603414, -275.6253767921893996, -332.2598985985115405 ) ) ;
#28763=CARTESIAN_POINT ( 'NONE',  ( -99.89363930626977606, -290.3416422727881923, -225.7358591512989960 ) ) ;
#28764=CARTESIAN_POINT ( 'NONE',  ( 21.14487628131042385, -292.5788476220254779, -315.3902543919811592 ) ) ;
#28765=CARTESIAN_POINT ( 'NONE',  ( -64.98618941442560981, -278.3680884398996227, -202.2654082010966476 ) ) ;
#28766=CARTESIAN_POINT ( 'NONE',  ( -55.57449699715751734, -295.9547298862773914, -198.3466138866595259 ) ) ;
#28767=CARTESIAN_POINT ( 'NONE',  ( -62.98840970067398359, -293.0262335022118805, -201.4881206174120791 ) ) ;
#28768=CARTESIAN_POINT ( 'NONE',  ( 10.64812456238589888, -278.9090924074130839, -330.4860931364851808 ) ) ;
#28769=CARTESIAN_POINT ( 'NONE',  ( -8.666708665526414279, -293.1636797723633094, -341.1309623486849318 ) ) ;
#28770=CARTESIAN_POINT ( 'NONE',  ( -34.52730176967966003, -290.6164701602526748, -344.1575610847003759 ) ) ;
#28771=CARTESIAN_POINT ( 'NONE',  ( -69.17788141322843387, -289.8790089403597676, -201.3510858327785229 ) ) ;
#28772=CARTESIAN_POINT ( 'NONE',  ( -0.6822781721375021924, -289.9805958015573992, -334.2277866984061916 ) ) ;
#28774=CARTESIAN_POINT ( 'NONE',  ( -39.95353643232859753, -289.8885107740105695, -343.5256460532460210 ) ) ;
#28776=CARTESIAN_POINT ( 'NONE',  ( -104.7990118038442660, -291.2854798970118395, -306.6587738163017320 ) ) ;
#28777=CARTESIAN_POINT ( 'NONE',  ( 2.963977390181769422, -278.6100219335698398, -206.6295460341603700 ) ) ;
#28778=CARTESIAN_POINT ( 'NONE',  ( -44.30020562026492570, -291.9618328155113431, -197.6427061757321439 ) ) ;
#28779=CARTESIAN_POINT ( 'NONE',  ( -111.3181032338351883, -279.1524250212343077, -249.0717761634805356 ) ) ;
#28780=CARTESIAN_POINT ( 'NONE',  ( 39.39097184169803256, -281.1419173055464285, -264.2095861541766908 ) ) ;
#28781=CARTESIAN_POINT ( 'NONE',  ( 35.66283086640006417, -285.3306234409656099, -253.1201032097440304 ) ) ;
#28783=CARTESIAN_POINT ( 'NONE',  ( 30.43264197193260401, -280.0943313019511720, -300.7775708613740449 ) ) ;
#28784=CARTESIAN_POINT ( 'NONE',  ( -111.9179442045474673, -282.4497652697301646, -278.3225542173382792 ) ) ;
#28786=CARTESIAN_POINT ( 'NONE',  ( -101.2994228653708149, -277.5846978210195175, -228.6468260384091309 ) ) ;
#28787=CARTESIAN_POINT ( 'NONE',  ( -39.18623166806359137, -298.9697291282907372, -197.1366063800762163 ) ) ;
#28789=CARTESIAN_POINT ( 'NONE',  ( -108.8890314041174321, -292.3891166012578537, -252.2149193404050607 ) ) ;
#28790=CARTESIAN_POINT ( 'NONE',  ( 38.79493661825399897, -277.0589217242993527, -276.8278665254196653 ) ) ;
#28791=CARTESIAN_POINT ( 'NONE',  ( 20.03644140286077402, -275.8560013074880999, -315.5458010475625770 ) ) ;
#28792=CARTESIAN_POINT ( 'NONE',  ( 21.27234464330004471, -296.1957981175326040, -317.1725655096025207 ) ) ;
#28793=CARTESIAN_POINT ( 'NONE',  ( -40.33663377911964432, -289.2554738408596791, -347.3159333614233333 ) ) ;
#28794=CARTESIAN_POINT ( 'NONE',  ( 28.49497332547324291, -280.1234953656467610, -307.5466164315567994 ) ) ;
#28795=CARTESIAN_POINT ( 'NONE',  ( -16.62457428114823443, -292.1459744064137567, -196.2004767964906762 ) ) ;
#28798=CARTESIAN_POINT ( 'NONE',  ( -93.61295820892578945, -290.2739778298624174, -223.4698693404680228 ) ) ;
#28799=CARTESIAN_POINT ( 'NONE',  ( 18.03529585480070807, -292.2587546086457451, -321.0172525842050959 ) ) ;
#28802=CARTESIAN_POINT ( 'NONE',  ( -9.698385558259470685, -291.9307939020596905, -202.6771470504879744 ) ) ;
#28805=CARTESIAN_POINT ( 'NONE',  ( 17.40634833298269157, -278.4094976428775681, -226.7417163044926838 ) ) ;
#28806=CARTESIAN_POINT ( 'NONE',  ( -114.1311705925976128, -295.5846797632743232, -272.4513884326486277 ) ) ;
#28807=CARTESIAN_POINT ( 'NONE',  ( -99.37870319314350809, -285.2687899150178055, -315.2235987037710174 ) ) ;
#28808=CARTESIAN_POINT ( 'NONE',  ( -68.77301236666075113, -285.4603964340911375, -204.4605120308521862 ) ) ;
#28809=CARTESIAN_POINT ( 'NONE',  ( 14.23023762699518535, -277.8320010408476151, -323.0729031931026611 ) ) ;
#28810=CARTESIAN_POINT ( 'NONE',  ( 33.08367019892872207, -291.8959899469087986, -295.2566704506836004 ) ) ;
#28811=CARTESIAN_POINT ( 'NONE',  ( 36.30124594681166172, -295.2096529922422405, -262.4719304339528207 ) ) ;
#28812=CARTESIAN_POINT ( 'NONE',  ( 35.01970173093855720, -274.1848892468259464, -257.9998794282258245 ) ) ;
#28815=CARTESIAN_POINT ( 'NONE',  ( -96.49789439135609825, -295.5559563336266251, -319.6389903965605868 ) ) ;
#28816=CARTESIAN_POINT ( 'NONE',  ( 36.18534113489588577, -289.6237193719618404, -282.0652704227585446 ) ) ;
#28817=CARTESIAN_POINT ( 'NONE',  ( 202.3298055824671451, 295.8616505545806490, -54.00000000005272227 ) ) ;
#28818=CARTESIAN_POINT ( 'NONE',  ( -35.49503363150593316, -299.1544289038358215, -193.6698978566819846 ) ) ;
#28820=CARTESIAN_POINT ( 'NONE',  ( -11.99440577218066650, -287.0423975113939719, -201.7943086867818749 ) ) ;
#28822=CARTESIAN_POINT ( 'NONE',  ( -59.22356883615201895, -278.8343923080984723, -196.7812020120217085 ) ) ;
#28823=CARTESIAN_POINT ( 'NONE',  ( -11.08420626853754243, -295.3702643978236893, -342.6938683094772955 ) ) ;
#28824=CARTESIAN_POINT ( 'NONE',  ( -79.86723194037270446, -287.7597614680824449, -333.1292517079456843 ) ) ;
#28825=CARTESIAN_POINT ( 'NONE',  ( -112.2547608864246058, -297.1070404181467666, -252.6473487767363224 ) ) ;
#28826=CARTESIAN_POINT ( 'NONE',  ( 33.79698566769963719, -294.1033403992008175, -286.8896772084623876 ) ) ;
#28830=CARTESIAN_POINT ( 'NONE',  ( 24.13311201855888299, -288.4663105816386519, -225.1554189438206208 ) ) ;
#28831=CARTESIAN_POINT ( 'NONE',  ( -37.37352853689063181, -292.5523547857346784, -350.3611179825600175 ) ) ;
#28832=CARTESIAN_POINT ( 'NONE',  ( -53.73065286795355178, -279.1958762765853521, -195.1753039448010725 ) ) ;
#28833=CARTESIAN_POINT ( 'NONE',  ( -99.02953988683130149, -285.9759625273129018, -312.8145669772147812 ) ) ;
#28834=CARTESIAN_POINT ( 'NONE',  ( -54.81212673754028941, -284.4065485833248772, -195.9743551455837860 ) ) ;
#28835=CARTESIAN_POINT ( 'NONE',  ( -37.29111180848410356, -287.1313613514339522, -344.8011048372808887 ) ) ;
#28836=CARTESIAN_POINT ( 'NONE',  ( 38.08518940720618673, -277.3149590415783905, -262.6816036032384432 ) ) ;
#28837=CARTESIAN_POINT ( 'NONE',  ( -108.5564594920096937, -273.0983046918013315, -254.2196950087486869 ) ) ;
#28839=CARTESIAN_POINT ( 'NONE',  ( -23.44187096779099733, -293.5556898561823687, -342.5798080740376577 ) ) ;
#28840=CARTESIAN_POINT ( 'NONE',  ( -108.2896682300805367, -278.7789122217877207, -253.1743258968416797 ) ) ;
#28841=CARTESIAN_POINT ( 'NONE',  ( -54.50869012156004345, -279.1744200107929146, -199.2512171389226410 ) ) ;
#28842=CARTESIAN_POINT ( 'NONE',  ( -1.458348260171868471, -275.5963164111367405, -202.5829683382581550 ) ) ;
#28843=CARTESIAN_POINT ( 'NONE',  ( -97.37609346310041758, -277.9871065381591961, -222.7808664332428918 ) ) ;
#28844=CARTESIAN_POINT ( 'NONE',  ( 191.8446247329872847, 278.1462026667327336, -124.7934328400877888 ) ) ;
#28845=CARTESIAN_POINT ( 'NONE',  ( -109.7812906963783206, -297.6688955621442574, -294.6739131878267131 ) ) ;
#28846=CARTESIAN_POINT ( 'NONE',  ( -112.3452863284742875, -275.1604526064900824, -261.9424758988611188 ) ) ;
#28848=CARTESIAN_POINT ( 'NONE',  ( -60.08753595986023299, -286.8299548504339782, -200.6699921097011270 ) ) ;
#28849=CARTESIAN_POINT ( 'NONE',  ( -112.8157800602518108, -286.4239573457176107, -261.5499165210116530 ) ) ;
#28850=CARTESIAN_POINT ( 'NONE',  ( 33.48938999505083558, -286.6618383989097083, -252.2315952118016185 ) ) ;
#28851=CARTESIAN_POINT ( 'NONE',  ( -99.74224886571371940, -283.4615606868936766, -315.4579204112681055 ) ) ;
#28852=CARTESIAN_POINT ( 'NONE',  ( -34.25974200469502762, -278.4913776758122594, -196.6128151678672396 ) ) ;
#28853=CARTESIAN_POINT ( 'NONE',  ( -14.20311892320789937, -288.2157255676131058, -199.7701866989403925 ) ) ;
#28854=CARTESIAN_POINT ( 'NONE',  ( 34.44009852084044354, -279.8141140215886935, -253.6853530091659366 ) ) ;
#28855=CARTESIAN_POINT ( 'NONE',  ( -76.60522581770916872, -278.9043858114934551, -332.5467947163360805 ) ) ;
#28856=CARTESIAN_POINT ( 'NONE',  ( 32.11836292259848591, -275.7421839848446439, -247.5425506151249806 ) ) ;
#28857=CARTESIAN_POINT ( 'NONE',  ( 21.17572012678067495, -287.0165468532685509, -319.7951168747990778 ) ) ;
#28858=CARTESIAN_POINT ( 'NONE',  ( -8.090866874796358132, -283.4816052470200134, -341.4706745622053177 ) ) ;
#28859=CARTESIAN_POINT ( 'NONE',  ( 15.71563345589393990, -282.8172484453177162, -326.0786758621821946 ) ) ;
#28862=CARTESIAN_POINT ( 'NONE',  ( 0.1293585361110431431, -290.4196608702520166, -336.2704337970289430 ) ) ;
#28863=CARTESIAN_POINT ( 'NONE',  ( -103.3812675367113485, -288.7298279289464062, -309.0933146043315674 ) ) ;
#28864=CARTESIAN_POINT ( 'NONE',  ( -35.13138682590787454, -297.2776836930663080, -197.1999511348621184 ) ) ;
#28865=CARTESIAN_POINT ( 'NONE',  ( 13.32242747412087702, -293.7140678336183441, -328.2802986577050319 ) ) ;
#28866=CARTESIAN_POINT ( 'NONE',  ( -91.11178114890505242, -288.3130445725331015, -320.8289745958236381 ) ) ;
#28867=CARTESIAN_POINT ( 'NONE',  ( 36.21137097158838714, -291.9050757092118147, -279.0514716277992306 ) ) ;
#28868=CARTESIAN_POINT ( 'NONE',  ( 35.38747543088187797, -288.6227525034599353, -260.1113101462957502 ) ) ;
#28869=CARTESIAN_POINT ( 'NONE',  ( -95.99890600148557951, -293.6948066931273615, -223.6242672951989618 ) ) ;
#28870=CARTESIAN_POINT ( 'NONE',  ( -6.426996150012344700, -290.6462704095212075, -338.6932607126948369 ) ) ;
#28871=CARTESIAN_POINT ( 'NONE',  ( -112.3565625322728465, -288.6131608099379378, -265.5863046297953360 ) ) ;
#28873=CARTESIAN_POINT ( 'NONE',  ( -31.77159710093684097, -294.1224870392187540, -195.5176157910393613 ) ) ;
#28874=CARTESIAN_POINT ( 'NONE',  ( -97.71955762335068130, -284.9172249295660322, -311.8973144673603883 ) ) ;
#28875=CARTESIAN_POINT ( 'NONE',  ( 29.26234011649155420, -295.0905173491903497, -235.4076358884279045 ) ) ;
#28878=CARTESIAN_POINT ( 'NONE',  ( -49.47969221070077595, -275.8781716099782670, -195.9372561731233304 ) ) ;
#28879=CARTESIAN_POINT ( 'NONE',  ( 35.19426935297148873, -280.6186970349644412, -260.4376077522010746 ) ) ;
#28880=CARTESIAN_POINT ( 'NONE',  ( -10.27718706193942033, -280.6989166951829020, -340.3626569397173398 ) ) ;
#28881=CARTESIAN_POINT ( 'NONE',  ( -110.6559660482669329, -296.0409708954169332, -247.1809637196172105 ) ) ;
#28882=CARTESIAN_POINT ( 'NONE',  ( 3.507644941049418819, -272.8492172630388382, -208.5802881947172125 ) ) ;
#28883=CARTESIAN_POINT ( 'NONE',  ( -108.5002517370127890, -276.3460535014623929, -292.3919735972970102 ) ) ;
#28884=CARTESIAN_POINT ( 'NONE',  ( -109.2652040852746325, -298.0660697193143278, -255.1924947416337943 ) ) ;
#28885=CARTESIAN_POINT ( 'NONE',  ( -18.04868583408125460, -296.2237972474559911, -341.3762890027979324 ) ) ;
#28887=CARTESIAN_POINT ( 'NONE',  ( -23.47823908267664450, -295.6733556268970915, -342.2488046534497244 ) ) ;
#28888=CARTESIAN_POINT ( 'NONE',  ( 129.8483263487583201, -299.5541904835127980, -201.6997734963854612 ) ) ;
#28889=CARTESIAN_POINT ( 'NONE',  ( -7.960660604380052519, -284.4551204923432692, -200.9142994269091673 ) ) ;
#28890=CARTESIAN_POINT ( 'NONE',  ( -106.7067850686869264, -296.8559767729030909, -247.4525667566919651 ) ) ;
#28891=CARTESIAN_POINT ( 'NONE',  ( -86.10237042656079609, -283.7070983024665907, -329.9547169009252912 ) ) ;
#28892=CARTESIAN_POINT ( 'NONE',  ( 38.65341023934551146, -287.3763871517948587, -282.9524159463294382 ) ) ;
#28893=CARTESIAN_POINT ( 'NONE',  ( -76.21172389521086643, -297.5484079566459172, -334.9782067397379706 ) ) ;
#28894=CARTESIAN_POINT ( 'NONE',  ( 37.24986043196271623, -291.6293351534392286, -276.3717350595569542 ) ) ;
#28895=CARTESIAN_POINT ( 'NONE',  ( -82.13641513467004529, -278.6553788043834743, -207.9304177820912969 ) ) ;
#28896=CARTESIAN_POINT ( 'NONE',  ( -4.829096099716524648, -292.1237833571632905, -337.9475929042657754 ) ) ;
#28898=CARTESIAN_POINT ( 'NONE',  ( 30.33381368716085191, -285.9663571425842861, -241.8189539107204951 ) ) ;
#28899=CARTESIAN_POINT ( 'NONE',  ( -106.2418717846092164, -289.0369085096439221, -304.1606323191239767 ) ) ;
#28902=CARTESIAN_POINT ( 'NONE',  ( -107.6249629562468755, -297.8550489476252210, -293.0364799822762052 ) ) ;
#28903=CARTESIAN_POINT ( 'NONE',  ( -67.14946832207321847, -281.0941991659597079, -200.0041478300858273 ) ) ;
#28904=CARTESIAN_POINT ( 'NONE',  ( -112.7215773493294506, -294.5462066957920229, -272.3995915035764597 ) ) ;
#28905=CARTESIAN_POINT ( 'NONE',  ( 22.59970398232882616, -281.7999614411745029, -312.0638224521202346 ) ) ;
#28906=CARTESIAN_POINT ( 'NONE',  ( -32.01039082659227830, -295.1533505007510030, -347.1895868161587941 ) ) ;
#28907=CARTESIAN_POINT ( 'NONE',  ( 23.55745648019969352, -285.0265905837824789, -225.6329733235589572 ) ) ;
#28908=CARTESIAN_POINT ( 'NONE',  ( -101.7085883252702558, -281.0687960868983737, -231.7645705731140993 ) ) ;
#28910=CARTESIAN_POINT ( 'NONE',  ( -90.20743865831647668, -296.3406560736297592, -219.6069813580631092 ) ) ;
#28913=CARTESIAN_POINT ( 'NONE',  ( -1.619842738583425090, -284.5561992301912824, -335.9180515230037827 ) ) ;
#28914=CARTESIAN_POINT ( 'NONE',  ( 128.9960186029002500, -299.5541904835127980, -189.6092331708328800 ) ) ;
#28915=CARTESIAN_POINT ( 'NONE',  ( -54.42813229853333468, -283.3380690714491266, -195.3538533559490702 ) ) ;
#28916=CARTESIAN_POINT ( 'NONE',  ( 3.407182085537348915, -275.7167100639817932, -335.5673362482120865 ) ) ;
#28917=CARTESIAN_POINT ( 'NONE',  ( -14.84438489160445585, -292.1852371359844369, -200.9142259596434883 ) ) ;
#28918=CARTESIAN_POINT ( 'NONE',  ( 35.83059945120395184, -283.1920351565196370, -279.5254299274858454 ) ) ;
#28919=CARTESIAN_POINT ( 'NONE',  ( 20.46960276339095586, -276.5115508354709277, -224.4683240407934761 ) ) ;
#28920=CARTESIAN_POINT ( 'NONE',  ( -27.45549092336016983, -284.5288100451078321, -345.9698869229168281 ) ) ;
#28921=CARTESIAN_POINT ( 'NONE',  ( 35.82350422358431530, -280.4315655279017392, -276.8011701266889872 ) ) ;
#28922=CARTESIAN_POINT ( 'NONE',  ( -110.5647853983429343, -280.7613765760755768, -254.0732343844262004 ) ) ;
#28923=CARTESIAN_POINT ( 'NONE',  ( -94.14669870041457500, -273.4260333062524069, -218.3590358660443087 ) ) ;
#28924=CARTESIAN_POINT ( 'NONE',  ( 37.59137671681521908, -275.6077516816897628, -288.1389085637092649 ) ) ;
#28925=CARTESIAN_POINT ( 'NONE',  ( 36.86177358847764651, -295.5490182836845179, -276.2905938707750124 ) ) ;
#28929=CARTESIAN_POINT ( 'NONE',  ( -30.72284203198544361, -293.1089005543605026, -345.8362542708027263 ) ) ;
#28930=CARTESIAN_POINT ( 'NONE',  ( -62.04461048427199188, -273.2297477483849093, -201.6024482632961110 ) ) ;
#28932=CARTESIAN_POINT ( 'NONE',  ( 30.27548918993041127, -294.6105560745963317, -234.8832662389708048 ) ) ;
#28933=CARTESIAN_POINT ( 'NONE',  ( -88.52914483777347243, -299.9090924074130271, -206.2264541496106460 ) ) ;
#28934=CARTESIAN_POINT ( 'NONE',  ( 3.914688565619278471, -293.7991844086780588, -205.7543195144860420 ) ) ;
#28935=CARTESIAN_POINT ( 'NONE',  ( 19.22774422849473908, -290.2339909411588792, -319.4277797221233186 ) ) ;
#28936=CARTESIAN_POINT ( 'NONE',  ( -109.3763318661992088, -276.8139732446758217, -250.0395553538179456 ) ) ;
#28937=CARTESIAN_POINT ( 'NONE',  ( -86.02895724524111642, -279.6528627423621742, -326.7398146488165480 ) ) ;
#28938=CARTESIAN_POINT ( 'NONE',  ( 36.97392133928026681, -291.5657582740174121, -265.2411900562795495 ) ) ;
#28939=CARTESIAN_POINT ( 'NONE',  ( 14.30178325449721477, -282.6287310706824769, -214.8524646059202894 ) ) ;
#28940=CARTESIAN_POINT ( 'NONE',  ( -69.15569715810329399, -282.4011002079937498, -336.4211440577749954 ) ) ;
#28942=CARTESIAN_POINT ( 'NONE',  ( -67.79705522980630406, -283.1299678863632607, -336.7279683861327726 ) ) ;
#28943=CARTESIAN_POINT ( 'NONE',  ( 10.61894207598172279, -281.7764719849806738, -210.4493539139551501 ) ) ;
#28944=CARTESIAN_POINT ( 'NONE',  ( -96.87356453975938564, -282.6969799694008998, -318.5892648632062105 ) ) ;
#28945=CARTESIAN_POINT ( 'NONE',  ( -106.1291973049916066, -279.0527584682786824, -304.5556003163956120 ) ) ;
#28946=CARTESIAN_POINT ( 'NONE',  ( 34.55429637435049273, -277.3996438837572214, -296.0840157304401146 ) ) ;
#28947=CARTESIAN_POINT ( 'NONE',  ( 30.91033621190086578, -296.2662352645559167, -285.9065529553535612 ) ) ;
#28950=CARTESIAN_POINT ( 'NONE',  ( 10.49848309132422131, -300.6511726817209365, -195.3447991607771144 ) ) ;
#28951=CARTESIAN_POINT ( 'NONE',  ( -86.20047067655202966, -275.7534441357573201, -326.8624646329412258 ) ) ;
#28952=CARTESIAN_POINT ( 'NONE',  ( -61.38942291493036407, -293.5043150331485435, -198.2246214958697408 ) ) ;
#28953=CARTESIAN_POINT ( 'NONE',  ( 27.24424671980931834, -293.3678520085264836, -304.7117541904410132 ) ) ;
#28954=CARTESIAN_POINT ( 'NONE',  ( -114.1901376725091808, -290.0132347255718628, -274.0819445104036731 ) ) ;
#28956=CARTESIAN_POINT ( 'NONE',  ( 38.64905473251574364, -292.2338358891450412, -278.8475973002811088 ) ) ;
#28957=CARTESIAN_POINT ( 'NONE',  ( -6.665582515039180755, -284.8616166645765020, -203.2248413037354169 ) ) ;
#28958=CARTESIAN_POINT ( 'NONE',  ( -96.10646393974624857, -293.0405384886427669, -225.0006945102907139 ) ) ;
#28959=CARTESIAN_POINT ( 'NONE',  ( -41.34138630994763020, -284.4807912425298468, -196.7637859125881619 ) ) ;
#28960=CARTESIAN_POINT ( 'NONE',  ( -34.81290807134679710, -284.3349348120583500, -343.8232720601941423 ) ) ;
#28961=CARTESIAN_POINT ( 'NONE',  ( -20.53620572476283002, -289.7828224393147707, -345.3181941518132589 ) ) ;
#28962=CARTESIAN_POINT ( 'NONE',  ( -5.537367688399023713, -280.9745577941933448, -204.5851886470320835 ) ) ;
#28964=CARTESIAN_POINT ( 'NONE',  ( 38.83300420412186327, -292.2392755668338395, -261.7856932072620566 ) ) ;
#28965=CARTESIAN_POINT ( 'NONE',  ( 14.50231543153340041, -289.1478536772306143, -327.1461622820708612 ) ) ;
#28966=CARTESIAN_POINT ( 'NONE',  ( -1.823553757975173717, -289.0866774293936032, -338.6105735251213673 ) ) ;
#28967=CARTESIAN_POINT ( 'NONE',  ( -12.02397293614165008, -286.5577425152166597, -201.8920542067419035 ) ) ;
#28969=CARTESIAN_POINT ( 'NONE',  ( 144.2857639756989272, -299.5541904835127980, -195.3611179825600175 ) ) ;
#28970=CARTESIAN_POINT ( 'NONE',  ( -44.65246856521751795, -297.0040102630856040, -345.8249270846321224 ) ) ;
#28971=CARTESIAN_POINT ( 'NONE',  ( -111.1209207622825801, -294.9817350258296642, -290.6077195803351287 ) ) ;
#28972=CARTESIAN_POINT ( 'NONE',  ( -110.1989010009386760, -277.7150034526537752, -262.4437083242016229 ) ) ;
#28973=CARTESIAN_POINT ( 'NONE',  ( -41.18341899833677644, -273.5128063552895696, -193.4664108989695706 ) ) ;
#28974=CARTESIAN_POINT ( 'NONE',  ( -38.37121490453610306, -293.5451649047367937, -344.0472622282470638 ) ) ;
#28975=CARTESIAN_POINT ( 'NONE',  ( 16.16406211547253591, -276.5839931826102998, -219.1488325899674692 ) ) ;
#28976=CARTESIAN_POINT ( 'NONE',  ( -62.42514791531172591, -271.8618995807586316, -200.4920538214416865 ) ) ;
#28977=CARTESIAN_POINT ( 'NONE',  ( 28.75879494706067163, -295.1880379515787354, -302.3822187649667512 ) ) ;
#28978=CARTESIAN_POINT ( 'NONE',  ( -15.48762485314155590, -295.8423641450490891, -340.3904097115009222 ) ) ;
#28980=CARTESIAN_POINT ( 'NONE',  ( -111.9518616527507504, -294.6689553754105191, -261.2313741163425220 ) ) ;
#28981=CARTESIAN_POINT ( 'NONE',  ( -26.23635635124255572, -298.8391810069481949, -193.4618585974712346 ) ) ;
#28982=CARTESIAN_POINT ( 'NONE',  ( -95.34082787328908637, -275.2080839381553687, -222.7899847489195508 ) ) ;
#28983=CARTESIAN_POINT ( 'NONE',  ( -103.0512861727144696, -291.0566334374165081, -302.6977651373611025 ) ) ;
#28984=CARTESIAN_POINT ( 'NONE',  ( -0.7436776325022109724, -294.8852612765637105, -333.6064252522456854 ) ) ;
#28985=CARTESIAN_POINT ( 'NONE',  ( -108.0712897170277955, -280.8694747177243016, -244.2154874713867230 ) ) ;
#28986=CARTESIAN_POINT ( 'NONE',  ( -106.9633565252325269, -277.6464864830326746, -238.5141826871370938 ) ) ;
#28987=CARTESIAN_POINT ( 'NONE',  ( -5.505300626159884025, -281.9928251520344702, -340.3593783448894214 ) ) ;
#28988=CARTESIAN_POINT ( 'NONE',  ( 31.76003758802262311, -275.3358754356679015, -304.2205244116261724 ) ) ;
#28989=CARTESIAN_POINT ( 'NONE',  ( -42.35684137575063346, -278.3897723389686121, -194.3263313773717300 ) ) ;
#28990=CARTESIAN_POINT ( 'NONE',  ( -76.51480461952797896, -277.5296757884241288, -206.1487385595294768 ) ) ;
#28992=CARTESIAN_POINT ( 'NONE',  ( -84.37769171075041186, -296.0741399835027323, -213.8247033711687664 ) ) ;
#28993=CARTESIAN_POINT ( 'NONE',  ( -17.16330074450739218, -276.3126586687073427, -198.0734089972396816 ) ) ;
#28996=CARTESIAN_POINT ( 'NONE',  ( -19.74583758605215422, -290.2972542834143610, -197.0354181444677977 ) ) ;
#28997=CARTESIAN_POINT ( 'NONE',  ( -108.7984607606721568, -290.1880890298560871, -299.0478982113800726 ) ) ;
#28998=CARTESIAN_POINT ( 'NONE',  ( -24.49852348394544421, -276.2157303263848576, -196.2469100033235065 ) ) ;
#28999=CARTESIAN_POINT ( 'NONE',  ( -106.2062619362709057, -270.9421275431236609, -240.5198000244643026 ) ) ;
#29000=CARTESIAN_POINT ( 'NONE',  ( -111.5625583934719316, -284.0010943134173544, -250.2759955948271511 ) ) ;
#29003=CARTESIAN_POINT ( 'NONE',  ( -110.8748008331861428, -282.3616430174290031, -285.1860755719627605 ) ) ;
#29005=CARTESIAN_POINT ( 'NONE',  ( 26.58791597075114410, -291.8549687587049561, -234.1999249923817956 ) ) ;
#29006=CARTESIAN_POINT ( 'NONE',  ( -95.91733887330151731, -283.3238627160918668, -224.7360988177030094 ) ) ;
#29009=CARTESIAN_POINT ( 'NONE',  ( 36.01866949154955932, -291.7530438872581726, -286.0193155949615971 ) ) ;
#29010=CARTESIAN_POINT ( 'NONE',  ( -73.96043540945811401, -282.0089730032079842, -337.3661485315952291 ) ) ;
#29011=CARTESIAN_POINT ( 'NONE',  ( -67.10683697970357287, -279.0491425883923284, -337.8924221682263465 ) ) ;
#29012=CARTESIAN_POINT ( 'NONE',  ( -46.47346337248296066, -287.1437782387467905, -194.3044311099714889 ) ) ;
#29013=CARTESIAN_POINT ( 'NONE',  ( 34.28415687976975335, -287.7389726811379091, -284.5231338214018706 ) ) ;
#29014=CARTESIAN_POINT ( 'NONE',  ( -69.49259107951876047, -278.9090272880847579, -336.5694392468197975 ) ) ;
#29015=CARTESIAN_POINT ( 'NONE',  ( -100.7176125718345361, -278.8536731337037509, -307.0154808950087499 ) ) ;
#29016=CARTESIAN_POINT ( 'NONE',  ( -86.45986791267628746, -287.3706700735061190, -213.6142503674073510 ) ) ;
#29018=CARTESIAN_POINT ( 'NONE',  ( -68.17550808821938801, -297.4917492424456782, -199.7474200918037184 ) ) ;
#29019=CARTESIAN_POINT ( 'NONE',  ( -56.46314082938407353, -291.2795465154296721, -342.5689762963320391 ) ) ;
#29021=CARTESIAN_POINT ( 'NONE',  ( 44.71564893372296723, -284.0519495502702512, -270.3284710469131937 ) ) ;
#29023=CARTESIAN_POINT ( 'NONE',  ( 35.59791381397667465, -292.2337612449141488, -292.5908475678988339 ) ) ;
#29024=CARTESIAN_POINT ( 'NONE',  ( 35.24695587551692455, -288.9024075812861838, -257.3617023465223497 ) ) ;
#29025=CARTESIAN_POINT ( 'NONE',  ( -32.92462837685746990, -281.8687089084618265, -196.4797029203458578 ) ) ;
#29026=CARTESIAN_POINT ( 'NONE',  ( 20.14170289193872065, -289.6638870726213781, -320.7223159298603719 ) ) ;
#29027=CARTESIAN_POINT ( 'NONE',  ( 2.934854232252313455, -289.8390752478499621, -335.4701596716221275 ) ) ;
#29028=CARTESIAN_POINT ( 'NONE',  ( -86.14440799429006290, -285.7291711685608675, -327.3110639944490003 ) ) ;
#29029=CARTESIAN_POINT ( 'NONE',  ( -113.7173849210784340, -278.8462860324142980, -260.1699688639847068 ) ) ;
#29031=CARTESIAN_POINT ( 'NONE',  ( -44.68056695131800637, -293.2240498334932113, -345.6162875106165302 ) ) ;
#29032=CARTESIAN_POINT ( 'NONE',  ( 34.32520115508302894, -281.0268715361618774, -242.0578943965372503 ) ) ;
#29033=CARTESIAN_POINT ( 'NONE',  ( -107.4810670066979270, -274.7305812070057414, -246.0437436730007335 ) ) ;
#29035=CARTESIAN_POINT ( 'NONE',  ( -110.4542110544635705, -292.8376638359844719, -287.0812184334320705 ) ) ;
#29036=CARTESIAN_POINT ( 'NONE',  ( -63.19103103557907275, -271.9598535799216847, -198.9063343454448045 ) ) ;
#29037=CARTESIAN_POINT ( 'NONE',  ( -70.96441198728437882, -279.1036397310989514, -205.4817611755388782 ) ) ;
#29038=CARTESIAN_POINT ( 'NONE',  ( 20.53039896733878322, -277.4390960191549311, -320.5689112606822846 ) ) ;
#29039=CARTESIAN_POINT ( 'NONE',  ( -52.77624482539867046, -299.2759051960790657, -198.3563983033112663 ) ) ;
#29040=CARTESIAN_POINT ( 'NONE',  ( -99.60468865110435388, -283.0127284061310888, -315.3514211874347097 ) ) ;
#29041=CARTESIAN_POINT ( 'NONE',  ( -103.7448378495758732, -291.8753908846409217, -303.0505247013063581 ) ) ;
#29042=CARTESIAN_POINT ( 'NONE',  ( -37.62469496349078213, -299.5687839072248266, -194.0549736053249319 ) ) ;
#29043=CARTESIAN_POINT ( 'NONE',  ( -112.2156779358013807, -297.9613861491866373, -254.1166292051446192 ) ) ;
#29044=CARTESIAN_POINT ( 'NONE',  ( -41.10660323687478979, -297.0997811996043652, -345.1125715942354759 ) ) ;
#29045=CARTESIAN_POINT ( 'NONE',  ( -95.73109890873644190, -281.9066092731093818, -317.1864960370452309 ) ) ;
#29046=CARTESIAN_POINT ( 'NONE',  ( -113.1504587761377962, -290.3861378248961387, -256.9903886155433952 ) ) ;
#29047=CARTESIAN_POINT ( 'NONE',  ( -92.31723490415963340, -271.2811946360124011, -219.8492604868421552 ) ) ;
#29048=CARTESIAN_POINT ( 'NONE',  ( -57.56345499142655342, -287.3956018723699231, -196.8385141738557138 ) ) ;
#29050=CARTESIAN_POINT ( 'NONE',  ( -66.67518959869019568, -290.5789104255426878, -203.1765031529651537 ) ) ;
#29051=CARTESIAN_POINT ( 'NONE',  ( -88.93230042470179342, -231.1883730374851496, -347.8443031440752975 ) ) ;
#29053=CARTESIAN_POINT ( 'NONE',  ( -111.4188318680573531, -289.3637765323534836, -251.5685398234625438 ) ) ;
#29054=CARTESIAN_POINT ( 'NONE',  ( 22.76489284886658737, -287.7964449033113965, -311.8474175847650827 ) ) ;
#29056=CARTESIAN_POINT ( 'NONE',  ( -102.2641411289027644, -286.1685318409749925, -229.5374831143345489 ) ) ;
#29057=CARTESIAN_POINT ( 'NONE',  ( -43.20455690560347506, -277.4615066705574691, -343.1465175980730464 ) ) ;
#29059=CARTESIAN_POINT ( 'NONE',  ( 39.40230404837005551, -292.4720146818851845, -270.3238875060144437 ) ) ;
#29060=CARTESIAN_POINT ( 'NONE',  ( -88.24783923721381029, -284.3942640320466921, -328.0679437294831473 ) ) ;
#29061=CARTESIAN_POINT ( 'NONE',  ( -5.724965787271730555, -284.1640090736559046, -339.8095871122327480 ) ) ;
#29062=CARTESIAN_POINT ( 'NONE',  ( -99.76883797504858364, -284.2870556920759100, -315.4901381478383655 ) ) ;
#29063=CARTESIAN_POINT ( 'NONE',  ( 21.34343563640646124, -281.2761103640312967, -226.8873150514334043 ) ) ;
#29064=CARTESIAN_POINT ( 'NONE',  ( 161.7396164022935920, 220.2077545383955055, -205.3692606286431328 ) ) ;
#29066=CARTESIAN_POINT ( 'NONE',  ( 188.5613963121770951, 271.4186816058274871, -139.2599248928845554 ) ) ;
#29067=CARTESIAN_POINT ( 'NONE',  ( -13.84510484761940674, -91.62221105869700466, -356.6869422256752387 ) ) ;
#29068=CARTESIAN_POINT ( 'NONE',  ( -59.51486978482670764, -272.9548539942754246, -200.5875524095781088 ) ) ;
#29069=CARTESIAN_POINT ( 'NONE',  ( -33.44423038639822465, -294.5120093366608103, -347.2139082883693959 ) ) ;
#29070=CARTESIAN_POINT ( 'NONE',  ( -46.54096165037511668, -155.7550357926132563, -361.7467890835505386 ) ) ;
#29071=CARTESIAN_POINT ( 'NONE',  ( -73.69567043240977000, -272.2651325181229254, -202.9844239935560779 ) ) ;
#29072=CARTESIAN_POINT ( 'NONE',  ( -95.43246076348934537, -299.0543825337038584, -224.1406786409301617 ) ) ;
#29073=CARTESIAN_POINT ( 'NONE',  ( 35.48248658103275233, -288.7328330255010087, -260.0965237433304083 ) ) ;
#29075=CARTESIAN_POINT ( 'NONE',  ( -53.22880859076300908, -296.1921927033925499, -345.5182221984113653 ) ) ;
#29077=CARTESIAN_POINT ( 'NONE',  ( 26.41802359045723136, -287.5556859434273065, -234.5828957379837618 ) ) ;
#29078=CARTESIAN_POINT ( 'NONE',  ( -5.231116456524945946, -273.3852703353703077, -200.7162838074785327 ) ) ;
#29080=CARTESIAN_POINT ( 'NONE',  ( 1.696222031992290491, -295.3467683073545800, -336.5441932651527281 ) ) ;
#29081=CARTESIAN_POINT ( 'NONE',  ( -4.523087606019172036, -295.1235927253036380, -339.9634032918083335 ) ) ;
#29082=CARTESIAN_POINT ( 'NONE',  ( -110.1224613021566938, -290.6361096159917565, -276.6320202256051743 ) ) ;
#29084=CARTESIAN_POINT ( 'NONE',  ( -5.739231721537038311, -276.3846104338207397, -201.7273202418811024 ) ) ;
#29085=CARTESIAN_POINT ( 'NONE',  ( 29.60800248004706248, -273.8608169705200339, -233.0263933446041733 ) ) ;
#29087=CARTESIAN_POINT ( 'NONE',  ( -114.0183494559465345, -277.9727153105167190, -277.3192688016152943 ) ) ;
#29088=CARTESIAN_POINT ( 'NONE',  ( 7.836552397029881156, -273.0810117970672195, -212.0056048599940084 ) ) ;
#29089=CARTESIAN_POINT ( 'NONE',  ( -56.95749592203973322, -274.8729576808760839, -199.6721604216728849 ) ) ;
#29090=CARTESIAN_POINT ( 'NONE',  ( 22.66550013739908920, -277.0780269395269784, -312.4308675841695617 ) ) ;
#29091=CARTESIAN_POINT ( 'NONE',  ( 25.29638150318346490, -276.7367111557689441, -227.3212688693693337 ) ) ;
#29092=CARTESIAN_POINT ( 'NONE',  ( 35.29331601246170891, -273.8296556770546886, -290.4730998508809421 ) ) ;
#29093=CARTESIAN_POINT ( 'NONE',  ( -12.96644529667286605, -295.3784107777237296, -339.3328077123313733 ) ) ;
#29094=CARTESIAN_POINT ( 'NONE',  ( 34.01298760567167534, -292.3624934326741140, -288.3578803892060023 ) ) ;
#29096=CARTESIAN_POINT ( 'NONE',  ( -111.7663152143852017, -278.7995440758169821, -289.9193693193631702 ) ) ;
#29097=CARTESIAN_POINT ( 'NONE',  ( 18.99749941439776180, -275.0609477616424670, -223.9402756868155393 ) ) ;
#29098=CARTESIAN_POINT ( 'NONE',  ( -69.56974447718572208, -284.3216321490796759, -200.9591563923111721 ) ) ;
#29099=CARTESIAN_POINT ( 'NONE',  ( -100.0349930674739909, -299.1113143510482359, -228.8698566592242400 ) ) ;
#29101=CARTESIAN_POINT ( 'NONE',  ( -27.80540380412180568, -285.3735181291838217, -197.8238118626960045 ) ) ;
#29102=CARTESIAN_POINT ( 'NONE',  ( -104.0539731783285760, -276.3628978860571124, -302.5335886159700749 ) ) ;
#29103=CARTESIAN_POINT ( 'NONE',  ( -24.24240343840943623, -275.4564811043995860, -342.8269542996873724 ) ) ;
#29104=CARTESIAN_POINT ( 'NONE',  ( -76.02661583374984389, -285.5686600949732110, -334.6734646758580425 ) ) ;
#29105=CARTESIAN_POINT ( 'NONE',  ( 9.931441982945049318, -277.5887519358110467, -326.5071823024180162 ) ) ;
#29107=CARTESIAN_POINT ( 'NONE',  ( 11.29094710910536925, -273.1126274212361409, -211.6298916813352662 ) ) ;
#29108=CARTESIAN_POINT ( 'NONE',  ( 35.74464626691104741, -276.1836842788366084, -268.8516020120518419 ) ) ;
#29109=CARTESIAN_POINT ( 'NONE',  ( -17.50101914013604798, -282.3077298326380742, -197.8602503900464740 ) ) ;
#29111=CARTESIAN_POINT ( 'NONE',  ( 33.49558159549865621, -289.1335185447226763, -244.0667513925443473 ) ) ;
#29112=CARTESIAN_POINT ( 'NONE',  ( 34.77791310673228509, -291.2865290003802556, -249.7297042914721601 ) ) ;
#29114=CARTESIAN_POINT ( 'NONE',  ( -44.59312579435954405, -296.7534150013375438, -197.2724766090933883 ) ) ;
#29115=CARTESIAN_POINT ( 'NONE',  ( -108.1732005711365900, -288.9818407512015597, -248.0975386458894718 ) ) ;
#29116=CARTESIAN_POINT ( 'NONE',  ( -110.5532707284312579, -275.4615312476335589, -297.1751512281608143 ) ) ;
#29118=CARTESIAN_POINT ( 'NONE',  ( -20.66694027677849732, -287.3218445494675848, -344.8777644420810020 ) ) ;
#29119=CARTESIAN_POINT ( 'NONE',  ( -34.79878517241586167, -284.6198431166550904, -344.1298700032400575 ) ) ;
#29120=CARTESIAN_POINT ( 'NONE',  ( -66.77557355800242078, -283.9116180920170223, -200.3067026336862284 ) ) ;
#29121=CARTESIAN_POINT ( 'NONE',  ( -53.80396825775465430, -284.6927346109205246, -342.1378737106871313 ) ) ;
#29122=CARTESIAN_POINT ( 'NONE',  ( -108.8757939604941356, -285.1522222404969398, -285.7657808063830203 ) ) ;
#29123=CARTESIAN_POINT ( 'NONE',  ( -97.89818579242142960, -293.1414589367479948, -225.4917633979897005 ) ) ;
#29125=CARTESIAN_POINT ( 'NONE',  ( -73.93855528857008608, -273.9133214114679049, -202.5787884180904541 ) ) ;
#29127=CARTESIAN_POINT ( 'NONE',  ( -101.9712361042727053, -289.1538301272617559, -231.1152126964408922 ) ) ;
#29128=CARTESIAN_POINT ( 'NONE',  ( -91.32903597740350676, -277.7941952117706137, -325.3390414846945760 ) ) ;
#29129=CARTESIAN_POINT ( 'NONE',  ( 37.28745169635097056, -295.5729872885106602, -273.5342989218363527 ) ) ;
#29131=CARTESIAN_POINT ( 'NONE',  ( -37.37352853689063892, -294.5519495502701943, -195.3611179825600175 ) ) ;
#29132=CARTESIAN_POINT ( 'NONE',  ( -10.81328570904239328, -281.3837926511320688, -338.9532680287605899 ) ) ;
#29134=CARTESIAN_POINT ( 'NONE',  ( -95.25635016124610388, -277.2094317784462305, -222.6872571060159487 ) ) ;
#29135=CARTESIAN_POINT ( 'NONE',  ( -49.58870742807535947, -272.3787209193567946, -194.9903466706304869 ) ) ;
#29136=CARTESIAN_POINT ( 'NONE',  ( 26.72985948596472028, -274.4193969354574278, -235.0600287624716316 ) ) ;
#29138=CARTESIAN_POINT ( 'NONE',  ( 20.71728216863201055, -294.4383003060963802, -224.9549889925963555 ) ) ;
#29139=CARTESIAN_POINT ( 'NONE',  ( 13.05642461154988254, -293.7187528058617545, -217.2250899937149597 ) ) ;
#29140=CARTESIAN_POINT ( 'NONE',  ( 12.87746693168394074, -294.1625748489303760, -212.7708275576423489 ) ) ;
#29141=CARTESIAN_POINT ( 'NONE',  ( 38.73387060940101634, -294.7591191398213368, -261.7645859195664002 ) ) ;
#29142=CARTESIAN_POINT ( 'NONE',  ( -102.7691010398401232, -295.9452183478330767, -302.8521253715268244 ) ) ;
#29143=CARTESIAN_POINT ( 'NONE',  ( -106.9602979986835152, -292.1872567162244536, -298.3975410176632295 ) ) ;
#29144=CARTESIAN_POINT ( 'NONE',  ( -18.91633803435625794, -282.9881023005478369, -345.1790751643713406 ) ) ;
#29145=CARTESIAN_POINT ( 'NONE',  ( -27.13901650990876746, -272.3199669271991183, -195.2338429297683717 ) ) ;
#29146=CARTESIAN_POINT ( 'NONE',  ( 12.07920372808245801, -286.5505921830846887, -211.2443200335937092 ) ) ;
#29147=CARTESIAN_POINT ( 'NONE',  ( -84.01601927443815043, -279.6765865250532670, -328.6801328073227637 ) ) ;
#29148=CARTESIAN_POINT ( 'NONE',  ( -25.09069824947386707, -285.2708164133159130, -198.1063198607274671 ) ) ;
#29149=CARTESIAN_POINT ( 'NONE',  ( -40.28641619419729381, -287.0889835343469940, -345.3160326648110185 ) ) ;
#29150=CARTESIAN_POINT ( 'NONE',  ( -39.52749759425856269, -278.1646025339778134, -194.6150090660700300 ) ) ;
#29151=CARTESIAN_POINT ( 'NONE',  ( 175.8323451578035872, 256.8656992060370499, -165.6361338323774817 ) ) ;
#29152=CARTESIAN_POINT ( 'NONE',  ( -101.8284908261481689, -283.5909078835904324, -304.8118204259590698 ) ) ;
#29153=CARTESIAN_POINT ( 'NONE',  ( 26.40003754083123511, -283.3193200034374968, -312.8464048170004048 ) ) ;
#29154=CARTESIAN_POINT ( 'NONE',  ( 3.046116274273402258, -287.5830129726841733, -335.7047413454131402 ) ) ;
#29155=CARTESIAN_POINT ( 'NONE',  ( -111.6264491077817382, -280.3668226175572613, -253.3841780930724497 ) ) ;
#29156=CARTESIAN_POINT ( 'NONE',  ( -94.82910094152910574, -279.1797260664491205, -320.8437587737985837 ) ) ;
#29157=CARTESIAN_POINT ( 'NONE',  ( -105.5135257091426411, -278.7358286499509177, -244.1120337001885616 ) ) ;
#29158=CARTESIAN_POINT ( 'NONE',  ( -72.70881258811427017, -275.5616681384973390, -204.5690950504262275 ) ) ;
#29159=CARTESIAN_POINT ( 'NONE',  ( 39.44106649991496738, -293.4798670779348981, -264.5812608086622504 ) ) ;
#29160=CARTESIAN_POINT ( 'NONE',  ( -29.01410478942843341, -286.9661779110084012, -344.5399421679449006 ) ) ;
#29161=CARTESIAN_POINT ( 'NONE',  ( -79.17245378939333023, -293.0984648964697499, -206.6063663710047820 ) ) ;
#29163=CARTESIAN_POINT ( 'NONE',  ( -105.2534035761517544, -295.1042164483267811, -297.9695697255476716 ) ) ;
#29164=CARTESIAN_POINT ( 'NONE',  ( 29.50771087166731377, -293.6140288923708113, -299.7421277621942295 ) ) ;
#29165=CARTESIAN_POINT ( 'NONE',  ( -58.86515589873064869, -292.8597201375199575, -196.7524679427423280 ) ) ;
#29166=CARTESIAN_POINT ( 'NONE',  ( 2.752970255155656520, -281.2568265818979967, -209.1750191052834964 ) ) ;
#29168=CARTESIAN_POINT ( 'NONE',  ( -33.34066139994413902, -297.0214765620827393, -193.6709412598685844 ) ) ;
#29169=CARTESIAN_POINT ( 'NONE',  ( -74.37094452355594854, -290.1826304870281206, -337.7716094566268339 ) ) ;
#29170=CARTESIAN_POINT ( 'NONE',  ( -33.15113654118997744, -281.1395202298446634, -346.0228669787665012 ) ) ;
#29171=CARTESIAN_POINT ( 'NONE',  ( -99.00964989773964930, -290.2720389287857756, -316.4568578516767730 ) ) ;
#29172=CARTESIAN_POINT ( 'NONE',  ( -4.588881145092316594, -286.8293658582298349, -205.0974961436477315 ) ) ;
#29174=CARTESIAN_POINT ( 'NONE',  ( 82.97595463368493540, 83.32078986060837167, -300.5379249362064797 ) ) ;
#29175=CARTESIAN_POINT ( 'NONE',  ( -82.68567550127887955, -218.7616381193585369, -348.8841751239126552 ) ) ;
#29176=CARTESIAN_POINT ( 'NONE',  ( -109.4469695386476928, -277.5852997139115246, -282.8219877990129021 ) ) ;
#29177=CARTESIAN_POINT ( 'NONE',  ( -14.19830883110518727, -279.2796668975616967, -200.7473343617472210 ) ) ;
#29178=CARTESIAN_POINT ( 'NONE',  ( 39.68618914801349717, -275.2290613558049586, -271.1756566901154315 ) ) ;
#29179=CARTESIAN_POINT ( 'NONE',  ( 7.539219266477946491, -59.96618086862105912, -352.3314556225434444 ) ) ;
#29180=CARTESIAN_POINT ( 'NONE',  ( -111.8232840950418705, -277.3419118533252572, -253.2994666690804877 ) ) ;
#29181=CARTESIAN_POINT ( 'NONE',  ( -51.35076606621438344, -281.2521097727154142, -343.7322939613135304 ) ) ;
#29182=CARTESIAN_POINT ( 'NONE',  ( 35.40617110913215981, -295.5934885642024028, -292.4876899309440432 ) ) ;
#29183=CARTESIAN_POINT ( 'NONE',  ( -60.28423373526529616, -292.2390053195602491, -200.9421277696114885 ) ) ;
#29184=CARTESIAN_POINT ( 'NONE',  ( -97.76383482057222807, -288.6577371769941465, -312.2211252530668730 ) ) ;
#29185=CARTESIAN_POINT ( 'NONE',  ( 38.82207225999194122, -276.0708005949307449, -259.7595821425560416 ) ) ;
#29186=CARTESIAN_POINT ( 'NONE',  ( -109.8042172097347873, -296.5968520368127201, -279.6079501035316071 ) ) ;
#29191=CARTESIAN_POINT ( 'NONE',  ( -85.89841427233375271, -281.3061899865826376, -212.4002453333106644 ) ) ;
#29194=CARTESIAN_POINT ( 'NONE',  ( -38.37195606870359654, -281.1186155180223523, -197.0467910506306737 ) ) ;
#29195=CARTESIAN_POINT ( 'NONE',  ( -79.36923148431291963, -281.2537324225068005, -206.9919011014411296 ) ) ;
#29196=CARTESIAN_POINT ( 'NONE',  ( -29.43111246164405159, -282.0083793114825994, -343.2185905112864361 ) ) ;
#29197=CARTESIAN_POINT ( 'NONE',  ( 20.41082872211825716, -273.3918059169424737, -224.5658914370737023 ) ) ;
#29201=CARTESIAN_POINT ( 'NONE',  ( 22.52164770151876283, -277.0021341095891216, -318.5539008113069031 ) ) ;
#29203=CARTESIAN_POINT ( 'NONE',  ( 36.51795177621814759, -277.3840819300374392, -257.2589640638132664 ) ) ;
#29204=CARTESIAN_POINT ( 'NONE',  ( -34.33260792502838399, -275.5897465108141660, -346.7126186761420854 ) ) ;
#29207=CARTESIAN_POINT ( 'NONE',  ( -94.99526159398773473, -285.8641524627857962, -318.9039933696400908 ) ) ;
#29209=CARTESIAN_POINT ( 'NONE',  ( 33.93041027460741788, -292.9674106166887100, -286.9355972965731780 ) ) ;
#29210=CARTESIAN_POINT ( 'NONE',  ( -2.261994383531324093, -285.8526435615632408, -201.9159302307698454 ) ) ;
#29211=CARTESIAN_POINT ( 'NONE',  ( -81.24500300977861400, -281.8975713842697814, -330.0107499586101198 ) ) ;
#29212=CARTESIAN_POINT ( 'NONE',  ( -32.12187460345364798, -281.5597411000109673, -343.7649893997270851 ) ) ;
#29213=CARTESIAN_POINT ( 'NONE',  ( -7.658711325376004631, -284.5241356925522496, -202.0952086587204235 ) ) ;
#29214=CARTESIAN_POINT ( 'NONE',  ( 27.21152764206630437, -283.2312158833216245, -305.2897779658824220 ) ) ;
#29215=CARTESIAN_POINT ( 'NONE',  ( 25.27517611454112867, -272.9947051450940307, -229.0800392881023981 ) ) ;
#29216=CARTESIAN_POINT ( 'NONE',  ( -64.24547228200616189, -284.1067889720205244, -199.0545507684197162 ) ) ;
#29217=CARTESIAN_POINT ( 'NONE',  ( -110.0239771372214506, -298.3140285296810816, -288.9139008688837862 ) ) ;
#29219=CARTESIAN_POINT ( 'NONE',  ( -108.9925003029575805, -279.2941737878839490, -285.5127279019183106 ) ) ;
#29220=CARTESIAN_POINT ( 'NONE',  ( -8.080888646031574751, -288.4345302546277594, -201.0683073677778907 ) ) ;
#29225=CARTESIAN_POINT ( 'NONE',  ( 34.99832134895100211, -295.7534755775664621, -292.3613768722133273 ) ) ;
#29227=CARTESIAN_POINT ( 'NONE',  ( -112.2794960780222056, -276.5127736138019827, -273.4151946129711064 ) ) ;
#29228=CARTESIAN_POINT ( 'NONE',  ( -89.38962818188210235, -288.9604741283120006, -326.8869705227680811 ) ) ;
#29229=CARTESIAN_POINT ( 'NONE',  ( 6.522246961676673394, -292.8450356590520869, -329.7745567149770523 ) ) ;
#29230=CARTESIAN_POINT ( 'NONE',  ( -110.7735600908295623, -277.1976498108247142, -273.3620210332728675 ) ) ;
#29231=CARTESIAN_POINT ( 'NONE',  ( -99.46853136960000086, -295.2466248455440336, -229.6341334135434806 ) ) ;
#29232=CARTESIAN_POINT ( 'NONE',  ( -91.13146940179331068, -292.5827084799610134, -220.2635266549310984 ) ) ;
#29233=CARTESIAN_POINT ( 'NONE',  ( 31.95455697924148097, -277.6233781216988064, -236.9535640164627353 ) ) ;
#29234=CARTESIAN_POINT ( 'NONE',  ( 19.00451588280505533, -292.7387156367883563, -321.8949498740161062 ) ) ;
#29235=CARTESIAN_POINT ( 'NONE',  ( -56.25112352216549283, -290.8998438329404053, -341.7505921185205011 ) ) ;
#29236=CARTESIAN_POINT ( 'NONE',  ( -92.06652323086579770, -289.5240729087989848, -217.5684731567962729 ) ) ;
#29237=CARTESIAN_POINT ( 'NONE',  ( 34.59047430127931477, -289.1813606261325731, -285.9488803882938441 ) ) ;
#29239=CARTESIAN_POINT ( 'NONE',  ( -63.86993052914272084, -290.2098368975118774, -338.5979298408167324 ) ) ;
#29241=CARTESIAN_POINT ( 'NONE',  ( 18.36664193314086191, -289.4789523294811033, -322.9404803148823930 ) ) ;
#29242=CARTESIAN_POINT ( 'NONE',  ( -78.98046635984833586, -277.5143013959537370, -207.4923281208132266 ) ) ;
#29243=CARTESIAN_POINT ( 'NONE',  ( -11.52044663751431131, -280.7126117459726515, -197.7861401916131001 ) ) ;
#29244=CARTESIAN_POINT ( 'NONE',  ( 37.65786152474048976, -281.0012496004908940, -252.9593128452560222 ) ) ;
#29245=CARTESIAN_POINT ( 'NONE',  ( 22.76137158689731166, -286.1649596487548024, -315.2448564677266063 ) ) ;
#29247=CARTESIAN_POINT ( 'NONE',  ( 36.65827000853134621, -279.7763308771675383, -276.8828409284703866 ) ) ;
#29248=CARTESIAN_POINT ( 'NONE',  ( -67.66808405344656308, -283.6541095774777546, -201.7518474469312366 ) ) ;
#29249=CARTESIAN_POINT ( 'NONE',  ( -101.6168586613798226, -254.6069401012266837, -324.2417600373901791 ) ) ;
#29250=CARTESIAN_POINT ( 'NONE',  ( -95.36587843930522013, -277.7067649605712631, -220.7839922678124935 ) ) ;
#29251=CARTESIAN_POINT ( 'NONE',  ( -110.6265477432470448, -283.7595028859212789, -247.5810751916764332 ) ) ;
#29252=CARTESIAN_POINT ( 'NONE',  ( -52.69608049951457929, -298.7919627706066308, -198.7014422940439715 ) ) ;
#29253=CARTESIAN_POINT ( 'NONE',  ( -25.29839699456137225, -293.8082183287192493, -197.4983689543639400 ) ) ;
#29254=CARTESIAN_POINT ( 'NONE',  ( -111.8726039430083148, -274.1897108684652835, -253.5162175010727310 ) ) ;
#29255=CARTESIAN_POINT ( 'NONE',  ( 27.88207604144076157, -274.7734016328113285, -237.5290222701762559 ) ) ;
#29256=CARTESIAN_POINT ( 'NONE',  ( -7.160732329261499274, -296.6564308431242125, -339.0344453613610085 ) ) ;
#29257=CARTESIAN_POINT ( 'NONE',  ( -17.72227886142927034, -288.9725431679455596, -344.8196857477736330 ) ) ;
#29259=CARTESIAN_POINT ( 'NONE',  ( 33.23362328162392743, -279.9802170391257619, -297.3507071184428128 ) ) ;
#29260=CARTESIAN_POINT ( 'NONE',  ( 13.28007226992709633, -292.5708787839383263, -212.3401203716051668 ) ) ;
#29261=CARTESIAN_POINT ( 'NONE',  ( -37.53858739657136567, -291.1084099755564694, -197.1136035078857276 ) ) ;
#29262=AXIS2_PLACEMENT_3D ( 'NONE', #73373, #23157, #88488 ) ;
#29263=CARTESIAN_POINT ( 'NONE',  ( 20.72167270563129904, -292.2064658009685445, -317.8538452146927398 ) ) ;
#29267=CARTESIAN_POINT ( 'NONE',  ( -85.96531210550035951, -290.8645795948653472, -215.7610847968657595 ) ) ;
#29268=CARTESIAN_POINT ( 'NONE',  ( -4.884362290657007222, -287.4104553945318798, -200.7957427265180286 ) ) ;
#29269=CARTESIAN_POINT ( 'NONE',  ( -82.13390479932378696, -299.9090924074130271, -214.2458315076590907 ) ) ;
#29270=CARTESIAN_POINT ( 'NONE',  ( 1.639595032869546998, -293.6029651139949124, -336.4918887361526458 ) ) ;
#29271=CARTESIAN_POINT ( 'NONE',  ( -113.7148909600849720, -285.8001219697132456, -275.7001598946342256 ) ) ;
#29272=CARTESIAN_POINT ( 'NONE',  ( -83.64623087291148806, -285.2297540012796730, -213.8606071217083127 ) ) ;
#29274=CARTESIAN_POINT ( 'NONE',  ( -21.48514559712777938, -278.3654041614892094, -342.3808043153999279 ) ) ;
#29275=CARTESIAN_POINT ( 'NONE',  ( 35.03484017148956298, -291.8079632433044708, -288.6226409280334906 ) ) ;
#29276=CARTESIAN_POINT ( 'NONE',  ( 35.20536456878092224, -295.1215613726804463, -255.7017380611010253 ) ) ;
#29277=CARTESIAN_POINT ( 'NONE',  ( 32.89190705290275218, -274.6283159817035084, -291.7206337176042439 ) ) ;
#29280=CARTESIAN_POINT ( 'NONE',  ( 24.86668721480743827, -293.8210822821598072, -315.7249218374769271 ) ) ;
#29281=CARTESIAN_POINT ( 'NONE',  ( 25.46620039976995287, -290.0140475019359769, -310.3171166358277446 ) ) ;
#29282=CARTESIAN_POINT ( 'NONE',  ( -67.97253149468437528, -295.6499112059328240, -201.8875048730719186 ) ) ;
#29284=CARTESIAN_POINT ( 'NONE',  ( -86.18782160283986116, -296.7913387945891941, -329.4842854023831364 ) ) ;
#29285=CARTESIAN_POINT ( 'NONE',  ( -35.93981945779435705, -286.7216110189032747, -197.2726277867202214 ) ) ;
#29286=CARTESIAN_POINT ( 'NONE',  ( -111.6028824227297633, -277.3661766502970636, -289.8575166249461290 ) ) ;
#29287=CARTESIAN_POINT ( 'NONE',  ( -5.831873850135859350, -295.3000434646322105, -340.5069919516442951 ) ) ;
#29288=CARTESIAN_POINT ( 'NONE',  ( -3.631936701984918692, -286.7517272837823157, -338.2279774776856698 ) ) ;
#29289=CARTESIAN_POINT ( 'NONE',  ( -113.6310857095020737, -296.7519522179055116, -281.0311381682540173 ) ) ;
#29290=CARTESIAN_POINT ( 'NONE',  ( -102.4303384963426424, -291.3361796951817837, -237.1499812616203258 ) ) ;
#29293=CARTESIAN_POINT ( 'NONE',  ( 199.4771156391435909, 285.7106110357494799, -96.36288505264877813 ) ) ;
#29294=CARTESIAN_POINT ( 'NONE',  ( 26.54658699536406985, -288.5191017968975302, -228.6358915518084132 ) ) ;
#29295=CARTESIAN_POINT ( 'NONE',  ( 36.57525178469694538, -285.4809262143061801, -305.9938812882205070 ) ) ;
#29297=CARTESIAN_POINT ( 'NONE',  ( -111.2369941724989815, -278.1678896626916071, -249.0820600895909536 ) ) ;
#29298=CARTESIAN_POINT ( 'NONE',  ( -65.99468213782841985, -285.4280788798551498, -339.5056209625559518 ) ) ;
#29299=CARTESIAN_POINT ( 'NONE',  ( -110.5487124253690752, -282.8495047764516244, -292.3004167816417862 ) ) ;
#29300=CARTESIAN_POINT ( 'NONE',  ( -12.83645460561090346, -286.8109863193118372, -340.6519931993403247 ) ) ;
#29301=CARTESIAN_POINT ( 'NONE',  ( 37.91362374878300301, -277.5296628082317056, -279.5738039945867399 ) ) ;
#29303=CARTESIAN_POINT ( 'NONE',  ( -109.4226045148370474, -296.8872537692310516, -282.2914014885336655 ) ) ;
#29305=CARTESIAN_POINT ( 'NONE',  ( -15.46187376323332430, -293.4479043495455244, -340.5752933853732998 ) ) ;
#29306=CARTESIAN_POINT ( 'NONE',  ( -41.01184010622842635, -280.6585464203695324, -193.5375054045942704 ) ) ;
#29307=CARTESIAN_POINT ( 'NONE',  ( -97.99360814509853412, -279.1174730904012904, -229.6469081054717947 ) ) ;
#29308=CARTESIAN_POINT ( 'NONE',  ( -105.6065024531201288, -278.2511735350688582, -244.0696297045502661 ) ) ;
#29309=CARTESIAN_POINT ( 'NONE',  ( 37.64025098092676558, -276.4288790567144929, -254.1994124060468323 ) ) ;
#29310=CARTESIAN_POINT ( 'NONE',  ( -39.96620078074518290, -276.0047035939931561, -347.0201001841069228 ) ) ;
#29311=CARTESIAN_POINT ( 'NONE',  ( -100.2453943390851236, -246.1090379458852624, -332.2849923024065220 ) ) ;
#29312=CARTESIAN_POINT ( 'NONE',  ( -74.30528925763134396, -296.9585367403147984, -337.2956196989208024 ) ) ;
#29314=CARTESIAN_POINT ( 'NONE',  ( 82.62159395231145709, -301.6989411204110638, -194.0647457283005224 ) ) ;
#29315=CARTESIAN_POINT ( 'NONE',  ( -25.10369573999069104, -287.2914145170660163, -198.0291962984408372 ) ) ;
#29317=CARTESIAN_POINT ( 'NONE',  ( -96.80166308453296153, -286.9541282856457087, -223.0484682661965792 ) ) ;
#29318=CARTESIAN_POINT ( 'NONE',  ( -0.9478882906663393948, -287.9042454304174044, -333.8179859903800093 ) ) ;
#29319=CARTESIAN_POINT ( 'NONE',  ( 21.55885624896204789, -281.7268570729345925, -319.8611317393966260 ) ) ;
#29320=CARTESIAN_POINT ( 'NONE',  ( -109.2705305424456839, -276.7358167689553170, -286.9303279340336985 ) ) ;
#29321=CARTESIAN_POINT ( 'NONE',  ( -102.8502652135940423, -285.9432923757050276, -305.3917056556606440 ) ) ;
#29322=CARTESIAN_POINT ( 'NONE',  ( -101.4050829579864939, -277.5261855262379527, -233.9387247141416140 ) ) ;
#29323=CARTESIAN_POINT ( 'NONE',  ( -3.626410889033343743, -277.9125844165016019, -335.6644314573221095 ) ) ;
#29324=CARTESIAN_POINT ( 'NONE',  ( -0.5206695426793234160, -275.0480880899304452, -207.2418393351161967 ) ) ;
#29325=CARTESIAN_POINT ( 'NONE',  ( -29.03556492624219132, -287.7441644428831751, -346.5656431372566431 ) ) ;
#29326=CARTESIAN_POINT ( 'NONE',  ( -14.28597327597590372, -281.1464063719410547, -197.0073684124253930 ) ) ;
#29327=CARTESIAN_POINT ( 'NONE',  ( 23.35823728496385598, -282.6767960259183496, -317.6586672783503218 ) ) ;
#29331=CARTESIAN_POINT ( 'NONE',  ( -84.37897997720746446, -291.5516279490882425, -329.8233233905046404 ) ) ;
#29332=CARTESIAN_POINT ( 'NONE',  ( -97.78039800873339971, -288.6065142076912480, -317.2702010392779925 ) ) ;
#29333=CARTESIAN_POINT ( 'NONE',  ( -48.90079259854451976, -272.9601759853975977, -197.9924531407881716 ) ) ;
#29334=CARTESIAN_POINT ( 'NONE',  ( -98.26241506037216311, -290.5279766158877237, -223.4145625515403708 ) ) ;
#29335=CARTESIAN_POINT ( 'NONE',  ( -7.959686154167663119, -287.1400919220389483, -337.9982419961565938 ) ) ;
#29337=CARTESIAN_POINT ( 'NONE',  ( -34.80034623468725385, -290.3243715381823904, -196.3914246220124369 ) ) ;
#29338=CARTESIAN_POINT ( 'NONE',  ( 20.68075937321216529, -289.3870619719614297, -315.3317201925223685 ) ) ;
#29339=CARTESIAN_POINT ( 'NONE',  ( -54.49178911615187815, -294.3376638359846424, -195.3683826091709363 ) ) ;
#29341=CARTESIAN_POINT ( 'NONE',  ( 37.60706707357442724, -289.6027893337953287, -274.2920378283252489 ) ) ;
#29342=CARTESIAN_POINT ( 'NONE',  ( -67.56760762968578149, -289.6564177005360534, -201.5254206859607962 ) ) ;
#29343=CARTESIAN_POINT ( 'NONE',  ( -112.1069892527627019, -292.4682656310608877, -276.9071561157421115 ) ) ;
#29344=CARTESIAN_POINT ( 'NONE',  ( -85.00586868677645214, -284.6704331258662251, -325.9626960450234492 ) ) ;
#29345=CARTESIAN_POINT ( 'NONE',  ( 33.71106479835332692, -295.2337867547405494, -245.6775512770311707 ) ) ;
#29349=CIRCLE ( 'NONE', #88320, 2.397123461337413719 ) ;
#29350=CARTESIAN_POINT ( 'NONE',  ( 51.45114908912319862, -301.0756357822836549, -194.7723165178934721 ) ) ;
#29351=CARTESIAN_POINT ( 'NONE',  ( -21.36288250136400535, -282.0392451996212912, -341.8084761257622404 ) ) ;
#29352=CARTESIAN_POINT ( 'NONE',  ( -94.97486941952470829, -281.8891917100678484, -318.3550597851880752 ) ) ;
#29353=CARTESIAN_POINT ( 'NONE',  ( -111.4390201347630978, -295.4939936698626184, -290.7018649857376431 ) ) ;
#29354=CARTESIAN_POINT ( 'NONE',  ( 7.968710264204084126, -272.9210247110358409, -211.8381248859341781 ) ) ;
#29355=CARTESIAN_POINT ( 'NONE',  ( -96.43069591213753711, -276.0073951301653779, -315.6358877594307160 ) ) ;
#29356=CARTESIAN_POINT ( 'NONE',  ( -108.6575319309426533, -298.1006870904590755, -252.5529825906557733 ) ) ;
#29359=CARTESIAN_POINT ( 'NONE',  ( 33.69018346364105554, -295.2299990685132229, -289.6404662875638678 ) ) ;
#29361=CARTESIAN_POINT ( 'NONE',  ( -95.72702990780005905, -296.7367685734482166, -314.4697889355977622 ) ) ;
#29363=CARTESIAN_POINT ( 'NONE',  ( -86.65413264193442444, -283.3912579401395533, -213.3123178136127081 ) ) ;
#29364=CARTESIAN_POINT ( 'NONE',  ( -92.19067496786476568, -295.8644903838483629, -318.5336200872338281 ) ) ;
#29366=CARTESIAN_POINT ( 'NONE',  ( -107.9261298496792847, -284.9459327910967090, -239.4570626986516402 ) ) ;
#29367=CARTESIAN_POINT ( 'NONE',  ( 39.68124680641609814, -287.2338093497587010, -271.5551979139354444 ) ) ;
#29368=CARTESIAN_POINT ( 'NONE',  ( -34.76937862477920049, -290.0843910736490443, -195.5720038592361618 ) ) ;
#29369=CARTESIAN_POINT ( 'NONE',  ( -110.3929701802472891, -278.0515976507305140, -246.3664729343311990 ) ) ;
#29370=CARTESIAN_POINT ( 'NONE',  ( -110.4542110544635705, -276.2666405000204009, -253.6410175316879361 ) ) ;
#29372=AXIS2_PLACEMENT_3D ( 'NONE', #36486, #22732, #36957 ) ;
#29373=CARTESIAN_POINT ( 'NONE',  ( 34.08397165204494428, -286.5687793604742524, -287.2579791386397687 ) ) ;
#29374=CARTESIAN_POINT ( 'NONE',  ( -111.3309290714171311, -289.7267738329644544, -250.1349356681278948 ) ) ;
#29375=CARTESIAN_POINT ( 'NONE',  ( -86.44010706348282724, -280.8113878483986241, -211.7434181945305056 ) ) ;
#29376=CARTESIAN_POINT ( 'NONE',  ( -110.7102911236716096, -294.3518889388678872, -287.6058608085305650 ) ) ;
#29377=CARTESIAN_POINT ( 'NONE',  ( 35.37382106602651533, -281.1238157988054809, -263.1534771295596897 ) ) ;
#29378=CARTESIAN_POINT ( 'NONE',  ( 32.23093163559096297, -294.1430603046895271, -303.4800983943899837 ) ) ;
#29379=CARTESIAN_POINT ( 'NONE',  ( 4.404843850108581371, -284.6898753263513981, -207.3183114559111857 ) ) ;
#29380=CARTESIAN_POINT ( 'NONE',  ( -111.0359012744987552, -280.7321098370366030, -256.3579892542754806 ) ) ;
#29381=CARTESIAN_POINT ( 'NONE',  ( -105.1843630470213071, -295.2426135724037977, -297.9433864827450975 ) ) ;
#29384=CARTESIAN_POINT ( 'NONE',  ( 13.04512740545966487, -284.3239562838868437, -325.4339280745186898 ) ) ;
#29386=CARTESIAN_POINT ( 'NONE',  ( -114.2704648735229114, -282.0523547857346784, -270.3284710469133074 ) ) ;
#29387=CARTESIAN_POINT ( 'NONE',  ( -24.17719436905932895, -273.4131884429230581, -194.6046558516751190 ) ) ;
#29389=CARTESIAN_POINT ( 'NONE',  ( -110.3370706542666824, -290.3746258537798326, -271.1832409830090569 ) ) ;
#29390=CARTESIAN_POINT ( 'NONE',  ( 24.25147850832910379, -282.5154955652085391, -229.8094174413233759 ) ) ;
#29391=CARTESIAN_POINT ( 'NONE',  ( 7.804399590131722242, -276.2807535519903013, -211.9807266404847894 ) ) ;
#29392=CARTESIAN_POINT ( 'NONE',  ( 34.85771441707441909, -283.4642594479661852, -294.8908787054024287 ) ) ;
#29393=CARTESIAN_POINT ( 'NONE',  ( 34.45682094086119918, -280.1464296584865679, -255.0662503580414864 ) ) ;
#29394=CARTESIAN_POINT ( 'NONE',  ( -112.1554295852688341, -280.6201449716169805, -265.0784547196565768 ) ) ;
#29395=CARTESIAN_POINT ( 'NONE',  ( -9.110314918286391617, -298.3964705767396595, -193.3611128246564306 ) ) ;
#29396=CARTESIAN_POINT ( 'NONE',  ( -26.99441807673987626, -274.0134300104894578, -194.0060905329540901 ) ) ;
#29397=CARTESIAN_POINT ( 'NONE',  ( 21.67960775317680699, -296.0985604750633229, -315.7449705802935682 ) ) ;
#29400=CARTESIAN_POINT ( 'NONE',  ( 23.03015009568990834, -292.3115946483538323, -316.1382430998243080 ) ) ;
#29401=CARTESIAN_POINT ( 'NONE',  ( -32.68084841259125284, -273.6200948604792984, -197.4358600290842389 ) ) ;
#29403=CARTESIAN_POINT ( 'NONE',  ( -79.23013442843488008, -293.0184713644013641, -206.5165470158291612 ) ) ;
#29404=CARTESIAN_POINT ( 'NONE',  ( -115.3430155898818299, -299.2662352645559167, -252.5904736702033517 ) ) ;
#29405=CARTESIAN_POINT ( 'NONE',  ( 15.15482162060935245, -293.9782228119782417, -214.5018866470483658 ) ) ;
#29406=CARTESIAN_POINT ( 'NONE',  ( 25.05179979218134534, -290.1118196252296570, -311.7013548735850463 ) ) ;
#29407=CARTESIAN_POINT ( 'NONE',  ( -110.3909528865244170, -276.7617036368711751, -254.0595481132388329 ) ) ;
#29409=CARTESIAN_POINT ( 'NONE',  ( -36.42437046259212963, -278.9607565800590123, -344.8081824879960777 ) ) ;
#29410=CARTESIAN_POINT ( 'NONE',  ( 28.41893540962738740, -292.0993153451026387, -305.3546201167088157 ) ) ;
#29411=CARTESIAN_POINT ( 'NONE',  ( 16.95783756074546389, -284.1494412613818099, -323.2742158642019490 ) ) ;
#29413=CARTESIAN_POINT ( 'NONE',  ( -76.14195257550034057, -283.2526503301240837, -332.2806628266311009 ) ) ;
#29414=CARTESIAN_POINT ( 'NONE',  ( -77.34306858593862444, -280.6090111245109711, -204.8673559265859865 ) ) ;
#29415=CARTESIAN_POINT ( 'NONE',  ( -67.73797821593642254, -282.2372106319593286, -340.6752346150220774 ) ) ;
#29417=CARTESIAN_POINT ( 'NONE',  ( -45.61231619327399756, -278.0956526534120599, -346.7318830156660852 ) ) ;
#29419=CARTESIAN_POINT ( 'NONE',  ( -4.277598507016923790, -278.1443385272478395, -339.1466519217938753 ) ) ;
#29420=CARTESIAN_POINT ( 'NONE',  ( -53.35057174420112602, -294.3376638359845288, -200.3683826091709648 ) ) ;
#29422=CARTESIAN_POINT ( 'NONE',  ( -95.17157845193695209, -299.2114048752402482, -222.5843956695094050 ) ) ;
#29423=CARTESIAN_POINT ( 'NONE',  ( -110.6635947713711658, -276.3908901595825682, -284.4197173372234602 ) ) ;
#29424=CARTESIAN_POINT ( 'NONE',  ( -112.6647734145734461, -292.4441738851839432, -259.9546471555673293 ) ) ;
#29425=CARTESIAN_POINT ( 'NONE',  ( 14.38254807697182791, -293.6500238913429257, -322.0897589086158064 ) ) ;
#29426=CARTESIAN_POINT ( 'NONE',  ( 39.51652991492730393, -287.0030712347661392, -265.8282772508179050 ) ) ;
#29428=CARTESIAN_POINT ( 'NONE',  ( -34.89185439275038192, -293.5966742589454270, -346.7326084105980044 ) ) ;
#29429=CARTESIAN_POINT ( 'NONE',  ( -99.71799481791592257, -282.4117782820048319, -309.8984088639176093 ) ) ;
#29430=CARTESIAN_POINT ( 'NONE',  ( -56.35955021846258717, -291.1600894936623831, -342.1723946049600045 ) ) ;
#29431=CARTESIAN_POINT ( 'NONE',  ( -69.05593939818318461, -284.1071736670024279, -203.8271667218678829 ) ) ;
#29432=CARTESIAN_POINT ( 'NONE',  ( -15.97322681195358030, -284.0851011460346172, -340.6791940734782997 ) ) ;
#29433=CARTESIAN_POINT ( 'NONE',  ( -23.34304231179140743, -289.8187538933159431, -345.8926001683159939 ) ) ;
#29434=CARTESIAN_POINT ( 'NONE',  ( 0.4263973098515957960, -281.0621068020741404, -207.7600969120641707 ) ) ;
#29435=CARTESIAN_POINT ( 'NONE',  ( -32.05531119196263035, -293.7818161457046813, -346.7946078279915696 ) ) ;
#29437=CARTESIAN_POINT ( 'NONE',  ( 32.72183580609387832, -288.7587914706627998, -301.9088556574972131 ) ) ;
#29438=CARTESIAN_POINT ( 'NONE',  ( 36.72687429895443501, -288.3061303840279948, -291.2270650345608374 ) ) ;
#29439=CARTESIAN_POINT ( 'NONE',  ( -14.56801953567258856, -286.5222624954222397, -200.9513450132330377 ) ) ;
#29443=CARTESIAN_POINT ( 'NONE',  ( 14.64857673874188571, -296.1898147139193043, -325.4729732402030891 ) ) ;
#29445=CARTESIAN_POINT ( 'NONE',  ( -96.14321264268662048, -294.5742223207029156, -319.3271825074128287 ) ) ;
#29446=CARTESIAN_POINT ( 'NONE',  ( -95.79232511482905466, -278.2289813013987327, -226.2162438935023374 ) ) ;
#29448=CARTESIAN_POINT ( 'NONE',  ( 76.20810742708401619, -298.7873891220818336, -193.4751467522457915 ) ) ;
#29449=CARTESIAN_POINT ( 'NONE',  ( -0.4272579244908135676, -293.0321571942099013, -334.2004753444669518 ) ) ;
#29450=CARTESIAN_POINT ( 'NONE',  ( 28.75633267816644789, -276.8664871371324807, -237.0591049793897582 ) ) ;
#29451=CARTESIAN_POINT ( 'NONE',  ( -67.53861845606866154, -271.7913473142361909, -202.5311828194123223 ) ) ;
#29452=CARTESIAN_POINT ( 'NONE',  ( 34.71711950422785975, -294.9402849152867248, -284.3130719310346990 ) ) ;
#29453=CARTESIAN_POINT ( 'NONE',  ( 35.14573082668061232, -294.7799478305428238, -281.6369579766840729 ) ) ;
#29455=CARTESIAN_POINT ( 'NONE',  ( -90.32477271515504924, -295.3043287394883691, -217.0429930663200366 ) ) ;
#29456=CARTESIAN_POINT ( 'NONE',  ( -65.51240090560530405, -298.3448893561983937, -198.7519519267593466 ) ) ;
#29458=CARTESIAN_POINT ( 'NONE',  ( -48.08369117180302510, -290.1332854373709438, -342.8555095877779877 ) ) ;
#29459=CARTESIAN_POINT ( 'NONE',  ( -18.21087668178067531, -295.1319818954327161, -340.8316726912700574 ) ) ;
#29460=CARTESIAN_POINT ( 'NONE',  ( -90.15783077263444056, -279.7737683951879148, -324.1823107775127255 ) ) ;
#29461=CARTESIAN_POINT ( 'NONE',  ( -61.87354465805472614, -278.4247818858306687, -197.8381067584539039 ) ) ;
#29462=CARTESIAN_POINT ( 'NONE',  ( -70.43378196511422118, -282.8255107998761559, -339.7890100509052331 ) ) ;
#29463=CARTESIAN_POINT ( 'NONE',  ( 21.77781754669398850, -274.2384729107440080, -221.1859675820693951 ) ) ;
#29464=CARTESIAN_POINT ( 'NONE',  ( -98.73354046499858327, -282.0562806750648406, -312.5503565990406969 ) ) ;
#29465=CARTESIAN_POINT ( 'NONE',  ( -86.27522419327856085, -277.7864740231936480, -211.8804546012555932 ) ) ;
#29466=CARTESIAN_POINT ( 'NONE',  ( -39.50827033262464738, -278.0248805922515203, -195.2129372993834977 ) ) ;
#29468=CARTESIAN_POINT ( 'NONE',  ( -52.72205844680755149, -296.5358998172821998, -198.4431201703008014 ) ) ;
#29469=CARTESIAN_POINT ( 'NONE',  ( 8.542096661990747464, -278.4243122993293582, -329.7528266304913700 ) ) ;
#29471=CARTESIAN_POINT ( 'NONE',  ( 16.33606428778431052, -290.8294433668969532, -217.3999566058536459 ) ) ;
#29472=CARTESIAN_POINT ( 'NONE',  ( -91.59852996751116905, -289.7989041982640401, -325.0730742556975770 ) ) ;
#29473=CARTESIAN_POINT ( 'NONE',  ( -0.9557631166994403626, -276.5341259932836806, -204.5734499503155064 ) ) ;
#29474=CARTESIAN_POINT ( 'NONE',  ( -104.9985950553105312, -270.9780595309036926, -237.9953148188567127 ) ) ;
#29475=CARTESIAN_POINT ( 'NONE',  ( -114.1937163747865753, -283.7183314760066537, -272.8338147801064224 ) ) ;
#29477=CARTESIAN_POINT ( 'NONE',  ( -84.65766999013339955, -283.4005230564154090, -212.1038891505074560 ) ) ;
#29480=CARTESIAN_POINT ( 'NONE',  ( 36.10524484218158392, -292.3525312242224459, -270.7774077021125549 ) ) ;
#29481=CARTESIAN_POINT ( 'NONE',  ( -100.6505410521979229, -283.2182040647455210, -231.4965382461817853 ) ) ;
#29484=CARTESIAN_POINT ( 'NONE',  ( 37.53304326110730216, -291.4857647407284844, -265.2035058653610236 ) ) ;
#29485=CARTESIAN_POINT ( 'NONE',  ( -113.6326290101110743, -283.0728794613543187, -267.1243326976565413 ) ) ;
#29486=CARTESIAN_POINT ( 'NONE',  ( -16.13166826601583637, -278.3735794856958705, -341.1011678043516895 ) ) ;
#29487=CARTESIAN_POINT ( 'NONE',  ( -89.62649528327484916, -286.5398606072567418, -214.3040598409220081 ) ) ;
#29488=CARTESIAN_POINT ( 'NONE',  ( -104.5975538124137358, -284.9346704430700470, -241.8472131398092699 ) ) ;
#29491=CARTESIAN_POINT ( 'NONE',  ( -37.79531972675044216, -278.4831812290463517, -343.9615045579537878 ) ) ;
#29492=CARTESIAN_POINT ( 'NONE',  ( -99.61052880182131730, -279.8845740610955204, -231.8561862011571861 ) ) ;
#29493=CARTESIAN_POINT ( 'NONE',  ( -96.03168533942694296, -287.1941086566839658, -223.6654405631720977 ) ) ;
#29495=CARTESIAN_POINT ( 'NONE',  ( -34.85676911289912283, -294.8550630333614322, -347.3210109293037249 ) ) ;
#29496=CARTESIAN_POINT ( 'NONE',  ( -66.95896003704004329, -291.4219878731375957, -338.9339645148407385 ) ) ;
#29500=CARTESIAN_POINT ( 'NONE',  ( -99.90806341382572953, -287.6948066931273047, -220.5068182859052968 ) ) ;
#29501=CARTESIAN_POINT ( 'NONE',  ( 37.03484810655034210, -280.2375941489960383, -251.6629473883713501 ) ) ;
#29502=CARTESIAN_POINT ( 'NONE',  ( 37.81383276167081675, -292.1119220558337020, -283.0132909945513688 ) ) ;
#29503=CARTESIAN_POINT ( 'NONE',  ( 31.61659694450847624, -288.7270066686413088, -244.2275381038584499 ) ) ;
#29504=CARTESIAN_POINT ( 'NONE',  ( -41.12509386878392803, -281.7640248183469680, -196.4445437477745031 ) ) ;
#29505=CARTESIAN_POINT ( 'NONE',  ( 36.11965804806346370, -288.7096862772360168, -249.1487703829839120 ) ) ;
#29506=CARTESIAN_POINT ( 'NONE',  ( -109.3039150921467666, -286.2796852836164021, -291.5360506709352535 ) ) ;
#29507=CARTESIAN_POINT ( 'NONE',  ( -82.54456722724030726, -277.8176108042473516, -332.6965076942007613 ) ) ;
#29509=CARTESIAN_POINT ( 'NONE',  ( -33.68671046397255964, -296.1182331951688411, -195.7175501496955690 ) ) ;
#29510=CARTESIAN_POINT ( 'NONE',  ( 36.65675019654054267, -291.4364267330344660, -255.0154737681453696 ) ) ;
#29511=CARTESIAN_POINT ( 'NONE',  ( -28.22289647405976964, -279.9980152433248577, -193.8493513623973570 ) ) ;
#29512=CARTESIAN_POINT ( 'NONE',  ( -92.95903433394393289, -275.1033183609162052, -221.1922496042566877 ) ) ;
#29515=CARTESIAN_POINT ( 'NONE',  ( 21.31550574532285580, -284.6948066931273615, -317.0979686699210447 ) ) ;
#29516=CARTESIAN_POINT ( 'NONE',  ( -32.72152071888341851, -272.3494587132752258, -194.5020598458118855 ) ) ;
#29518=CARTESIAN_POINT ( 'NONE',  ( -108.6654609815782493, -278.2692726800484024, -254.4637435219671602 ) ) ;
#29519=CARTESIAN_POINT ( 'NONE',  ( 25.74862499282144768, -277.3348026351846443, -313.8996969709345422 ) ) ;
#29520=CARTESIAN_POINT ( 'NONE',  ( -44.64548351082566313, -299.3833389556023121, -197.0844480371542033 ) ) ;
#29521=CARTESIAN_POINT ( 'NONE',  ( -112.2979457114078770, -283.4031087708121390, -286.9255818186777560 ) ) ;
#29522=CARTESIAN_POINT ( 'NONE',  ( -96.56588323903820026, -291.6974498406003704, -314.7722385256952293 ) ) ;
#29523=CARTESIAN_POINT ( 'NONE',  ( -40.43174374055428189, -299.5342198424431785, -194.0653840559467369 ) ) ;
#29524=CARTESIAN_POINT ( 'NONE',  ( -33.37555111840804045, -299.3058391120957253, -193.7573961459067107 ) ) ;
#29525=CARTESIAN_POINT ( 'NONE',  ( 22.81505689442831297, -296.1610629426511991, -314.8717123808947349 ) ) ;
#29526=CARTESIAN_POINT ( 'NONE',  ( -100.5939507280918406, -282.0118106660077615, -310.4479420050581098 ) ) ;
#29527=CARTESIAN_POINT ( 'NONE',  ( -68.95677777649038376, -271.6545389789197316, -202.7280798775381641 ) ) ;
#29528=CARTESIAN_POINT ( 'NONE',  ( -0.1249202024432567587, -288.1388069382073809, -203.8529829890120482 ) ) ;
#29529=CARTESIAN_POINT ( 'NONE',  ( 20.59331829107336986, -287.1026851902126396, -315.3009178560034798 ) ) ;
#29530=CARTESIAN_POINT ( 'NONE',  ( -11.52259850706730937, -92.40725766065216362, -359.8631175693950581 ) ) ;
#29532=CARTESIAN_POINT ( 'NONE',  ( -80.22505478101170695, -288.1948350395160787, -333.6676294675148711 ) ) ;
#29533=CARTESIAN_POINT ( 'NONE',  ( -78.18975759646480128, -289.2847136255032297, -330.9490417433148082 ) ) ;
#29535=CARTESIAN_POINT ( 'NONE',  ( -68.38827364194628444, -286.7334435362445788, -200.2211765921711049 ) ) ;
#29536=CARTESIAN_POINT ( 'NONE',  ( -78.64046503454702020, -277.9584427451038664, -330.6431104899335764 ) ) ;
#29538=CARTESIAN_POINT ( 'NONE',  ( 24.57306022929602562, -291.8692496294517014, -225.1056767595034955 ) ) ;
#29539=CARTESIAN_POINT ( 'NONE',  ( -90.36184359896449791, -284.4300827330563379, -326.1313139827984173 ) ) ;
#29540=CARTESIAN_POINT ( 'NONE',  ( 27.72402831107037002, -283.5989735226227708, -310.3255460710678335 ) ) ;
#29541=CARTESIAN_POINT ( 'NONE',  ( -58.47686732894896977, -283.6512811276439834, -344.4371987148072094 ) ) ;
#29542=CARTESIAN_POINT ( 'NONE',  ( 9.286779929751507012, -281.0464595154438712, -214.1002583805804136 ) ) ;
#29543=CARTESIAN_POINT ( 'NONE',  ( 5.883814447466332531, -58.44289898758961499, -354.8377425840699289 ) ) ;
#29544=CARTESIAN_POINT ( 'NONE',  ( -99.14903296997707116, -279.9796998010316429, -312.5497661480141005 ) ) ;
#29545=CARTESIAN_POINT ( 'NONE',  ( 196.0938070543772653, 285.1859344014769704, -111.4769352986099022 ) ) ;
#29546=CARTESIAN_POINT ( 'NONE',  ( 63.78990005684839559, 47.06080592420466502, -315.5780313746797106 ) ) ;
#29547=CARTESIAN_POINT ( 'NONE',  ( -16.58508189228268392, -273.5243249269602188, -200.1530018079023989 ) ) ;
#29548=CARTESIAN_POINT ( 'NONE',  ( -66.90659241535628610, -294.9369876294423420, -341.4065981007842083 ) ) ;
#29549=CARTESIAN_POINT ( 'NONE',  ( 189.5630867786578051, 267.9798697570337254, -137.6296589465633247 ) ) ;
#29550=CARTESIAN_POINT ( 'NONE',  ( -100.7901325871747247, -271.8049220511685462, -227.5164554647896011 ) ) ;
#29551=CARTESIAN_POINT ( 'NONE',  ( -111.6196797160949785, -298.3977315625589881, -271.5054065634899985 ) ) ;
#29552=CARTESIAN_POINT ( 'NONE',  ( -42.68314824806152075, -290.4359842322951977, -343.7108522039593481 ) ) ;
#29554=CARTESIAN_POINT ( 'NONE',  ( -27.76526590967355190, -295.8747547571860537, -346.5792802118221516 ) ) ;
#29555=CARTESIAN_POINT ( 'NONE',  ( -30.53178661845068476, -286.6327936377331298, -197.5667993515575631 ) ) ;
#29556=CARTESIAN_POINT ( 'NONE',  ( -21.40555116452913609, -273.1722495103118149, -195.3442421139377245 ) ) ;
#29557=CARTESIAN_POINT ( 'NONE',  ( 37.26270513387246552, -294.1243896541595291, -251.9670554436861494 ) ) ;
#29558=CARTESIAN_POINT ( 'NONE',  ( -2.089625521674100650, -292.9985220296296689, -201.9590867474784659 ) ) ;
#29559=CARTESIAN_POINT ( 'NONE',  ( -57.65697699456558212, -291.9492503865397453, -200.1919834250715553 ) ) ;
#29561=CARTESIAN_POINT ( 'NONE',  ( -18.92507311505876544, -276.2074475718442272, -197.0258683489562088 ) ) ;
#29562=CARTESIAN_POINT ( 'NONE',  ( 4.658348096915016612, -273.4001194884110078, -206.2356692151504376 ) ) ;
#29565=CARTESIAN_POINT ( 'NONE',  ( -97.88436887837400491, -277.4246251232415261, -317.8386091141192082 ) ) ;
#29567=CARTESIAN_POINT ( 'NONE',  ( 36.40021857569557540, -274.0044083474932677, -274.3762493418935833 ) ) ;
#29568=CARTESIAN_POINT ( 'NONE',  ( -89.47160099107149733, -274.3757369873686116, -218.8179369648386228 ) ) ;
#29569=CARTESIAN_POINT ( 'NONE',  ( 35.34113345345461710, -276.6167951493111445, -279.7446308801069108 ) ) ;
#29570=CARTESIAN_POINT ( 'NONE',  ( -20.74755565520646527, -299.8567466513939053, -194.1566811824129957 ) ) ;
#29571=CARTESIAN_POINT ( 'NONE',  ( 36.87662076604977557, -273.4046722380957135, -257.2470163978131836 ) ) ;
#29572=CARTESIAN_POINT ( 'NONE',  ( -84.53759500551639405, -296.3734507739600303, -326.2526592484402386 ) ) ;
#29573=CARTESIAN_POINT ( 'NONE',  ( 33.31084321856834407, -292.3974848506645685, -290.9877463449442416 ) ) ;
#29575=CARTESIAN_POINT ( 'NONE',  ( -5.304678688281513566, -277.1341018165870764, -340.3122163352838925 ) ) ;
#29576=CARTESIAN_POINT ( 'NONE',  ( -0.5481045156054616951, -274.7224734834068158, -207.2970917509907167 ) ) ;
#29578=CARTESIAN_POINT ( 'NONE',  ( -113.8328822883666049, -283.2777944278572022, -267.1184951608079245 ) ) ;
#29579=CARTESIAN_POINT ( 'NONE',  ( -73.69677811966252534, -297.5333320837584097, -336.2094960699198509 ) ) ;
#29581=CARTESIAN_POINT ( 'NONE',  ( -102.3772737991617277, -284.2038733483617534, -236.8502856486077519 ) ) ;
#29583=CARTESIAN_POINT ( 'NONE',  ( -108.9473365334323347, -277.0364277085984099, -251.5868965467641942 ) ) ;
#29584=CARTESIAN_POINT ( 'NONE',  ( -102.3861380289366707, -276.6618199710036947, -304.7790786095912949 ) ) ;
#29585=CARTESIAN_POINT ( 'NONE',  ( -68.71584529783726225, -285.4646510790976777, -338.4973293159447962 ) ) ;
#29586=CARTESIAN_POINT ( 'NONE',  ( 17.57248324751267887, -276.0644018987672439, -221.5871324460565290 ) ) ;
#29588=CARTESIAN_POINT ( 'NONE',  ( 38.82280831909432095, -273.9983404106151852, -274.0260221535552887 ) ) ;
#29589=CARTESIAN_POINT ( 'NONE',  ( -64.11375111489769552, -281.7040289383692766, -200.0688658715786232 ) ) ;
#29591=CARTESIAN_POINT ( 'NONE',  ( -40.77596817475892266, -287.9295556933017224, -194.8279836521215600 ) ) ;
#29593=CARTESIAN_POINT ( 'NONE',  ( 37.40524269709768390, -291.6386379643914779, -277.1095863507511012 ) ) ;
#29594=CARTESIAN_POINT ( 'NONE',  ( 144.2857639756989272, -299.5541904835127980, -201.5153591320744226 ) ) ;
#29595=CARTESIAN_POINT ( 'NONE',  ( -83.48731640819566735, -272.0886817432012776, -213.1612440780648114 ) ) ;
#29596=CARTESIAN_POINT ( 'NONE',  ( -99.31791905587400038, -289.2501573249719513, -229.4044334768249769 ) ) ;
#29597=CARTESIAN_POINT ( 'NONE',  ( 143.8719904363247224, 176.7915900130879550, -240.1109971732525139 ) ) ;
#29598=CARTESIAN_POINT ( 'NONE',  ( -72.58284060742491306, -295.5854839513073671, -204.1418306257749009 ) ) ;
#29599=CARTESIAN_POINT ( 'NONE',  ( -113.1273492954476012, -288.9141755857889962, -279.7000315954782081 ) ) ;
#29600=CARTESIAN_POINT ( 'NONE',  ( -42.97385589386844629, -284.7244129787180782, -343.9965295405752386 ) ) ;
#29601=CARTESIAN_POINT ( 'NONE',  ( -37.95152406823138591, -284.2844759463075661, -194.3768950662571910 ) ) ;
#29602=CARTESIAN_POINT ( 'NONE',  ( -87.31577472453834332, -285.1902734362008118, -324.4490244565558896 ) ) ;
#29604=CARTESIAN_POINT ( 'NONE',  ( -73.86856342126864661, -284.3530359149967808, -333.8096173749000855 ) ) ;
#29605=CARTESIAN_POINT ( 'NONE',  ( -79.59698675849078597, -291.5994511851951074, -332.8172295792726914 ) ) ;
#29606=CARTESIAN_POINT ( 'NONE',  ( -70.12662235580337722, -273.9652705430538617, -200.6983546470103761 ) ) ;
#29607=CARTESIAN_POINT ( 'NONE',  ( -51.44103206270705186, -287.3109468979891972, -344.5940152338362168 ) ) ;
#29608=CARTESIAN_POINT ( 'NONE',  ( 26.06688202920612341, -276.1299213946431905, -314.1380885840816291 ) ) ;
#29609=CARTESIAN_POINT ( 'NONE',  ( -17.76539404128532240, -296.7783278587023688, -342.3931597405695015 ) ) ;
#29611=CARTESIAN_POINT ( 'NONE',  ( -54.42813229853333468, -291.7662352645558599, -345.3683826091709648 ) ) ;
#29612=CARTESIAN_POINT ( 'NONE',  ( -70.45200056094631691, -282.1828846080255744, -335.9873214110297681 ) ) ;
#29613=CARTESIAN_POINT ( 'NONE',  ( -81.49055733870788742, -275.6511190922333867, -331.1961969318503520 ) ) ;
#29614=CARTESIAN_POINT ( 'NONE',  ( -112.8552825989664115, -271.1750533094028128, -259.0283548681853745 ) ) ;
#29615=CARTESIAN_POINT ( 'NONE',  ( 27.95605332482075056, -274.4553207953253491, -237.4963030304643610 ) ) ;
#29616=CARTESIAN_POINT ( 'NONE',  ( 23.90683462294566652, -294.5085036339241924, -229.3815530336137272 ) ) ;
#29617=CARTESIAN_POINT ( 'NONE',  ( 33.53289891645359688, -294.2506797210995160, -251.9166158477855788 ) ) ;
#29618=CARTESIAN_POINT ( 'NONE',  ( -102.6550473413429927, -285.8430338034438023, -305.2859476292934460 ) ) ;
#29619=CARTESIAN_POINT ( 'NONE',  ( 6.145874232696984407, -294.0550847829957206, -207.5324846392213658 ) ) ;
#29620=CARTESIAN_POINT ( 'NONE',  ( 12.94168331329148280, -294.0524942904685304, -212.6993488351442636 ) ) ;
#29621=CARTESIAN_POINT ( 'NONE',  ( -98.73445341626768368, -295.8377693647446449, -309.9496714945110512 ) ) ;
#29622=CARTESIAN_POINT ( 'NONE',  ( -110.8952903346242351, -292.3632559662616472, -285.0851424638776166 ) ) ;
#29623=CARTESIAN_POINT ( 'NONE',  ( -13.41992111698593781, -282.9165543405028416, -343.5509293871369891 ) ) ;
#29624=CARTESIAN_POINT ( 'NONE',  ( -69.58423332470269429, -271.7719288451023090, -201.7851074256025186 ) ) ;
#29625=CARTESIAN_POINT ( 'NONE',  ( -33.72520494221807752, -285.9298046426694100, -193.4460936564299800 ) ) ;
#29626=CARTESIAN_POINT ( 'NONE',  ( -93.95808570444467023, -279.8546664687211774, -319.0071012647097746 ) ) ;
#29627=CARTESIAN_POINT ( 'NONE',  ( -60.08719069992943673, -284.5455757794537703, -200.5773579602496000 ) ) ;
#29628=CARTESIAN_POINT ( 'NONE',  ( 37.70092827517243705, -285.5671982561229925, -271.5457951417682807 ) ) ;
#29629=CARTESIAN_POINT ( 'NONE',  ( -73.16043522044930114, -277.7221382641683363, -203.5832180051226032 ) ) ;
#29630=CARTESIAN_POINT ( 'NONE',  ( -75.31871349344845612, -193.4224457575235192, -358.3059354159982490 ) ) ;
#29631=CARTESIAN_POINT ( 'NONE',  ( -108.9880835656874751, -284.2484207508248346, -256.0508355904121913 ) ) ;
#29632=CARTESIAN_POINT ( 'NONE',  ( 18.85836328065643386, -282.0444514180719011, -218.3076686106557247 ) ) ;
#29633=CARTESIAN_POINT ( 'NONE',  ( -7.023918916874150931, -287.7227311347126033, -340.8994394802101056 ) ) ;
#29634=CARTESIAN_POINT ( 'NONE',  ( -17.54588820591202136, -278.4010216360529171, -343.9448542552958656 ) ) ;
#29635=CARTESIAN_POINT ( 'NONE',  ( -42.75445766322408758, -278.4342814747827788, -346.6762562500495051 ) ) ;
#29636=CARTESIAN_POINT ( 'NONE',  ( -91.29538787645398656, -279.0905971059065109, -221.1879588114905175 ) ) ;
#29637=CARTESIAN_POINT ( 'NONE',  ( -2.160214114160412091, -276.5002122664850503, -204.5271613436518123 ) ) ;
#29638=CARTESIAN_POINT ( 'NONE',  ( 21.31044597694716813, -292.8793304468553629, -220.4518400622679053 ) ) ;
#29639=CARTESIAN_POINT ( 'NONE',  ( 11.16540628403935465, -286.3970434720236540, -327.1648582220523735 ) ) ;
#29641=CARTESIAN_POINT ( 'NONE',  ( -3.693172007110046007, -294.0888342864424772, -201.9784882843183595 ) ) ;
#29642=CARTESIAN_POINT ( 'NONE',  ( 28.66692138427277214, -292.9036584168970307, -302.3699572380102722 ) ) ;
#29643=CARTESIAN_POINT ( 'NONE',  ( -5.536134208376211951, -294.2885853628543487, -336.1053927999683424 ) ) ;
#29644=CARTESIAN_POINT ( 'NONE',  ( -79.43628431113995703, -292.5780917485774353, -206.1919484113753924 ) ) ;
#29645=CARTESIAN_POINT ( 'NONE',  ( 35.45303499439760486, -282.1083515570405780, -263.1330287051370078 ) ) ;
#29647=CARTESIAN_POINT ( 'NONE',  ( -108.9427853834417022, -271.9642400710333163, -242.5362613821383775 ) ) ;
#29648=CARTESIAN_POINT ( 'NONE',  ( -28.98000735492000857, -289.6003541596352875, -346.8566749568366276 ) ) ;
#29649=CARTESIAN_POINT ( 'NONE',  ( -66.12922475595220817, -281.5644939876680724, -340.4577718518989968 ) ) ;
#29650=CARTESIAN_POINT ( 'NONE',  ( -31.82405520611115435, -289.3177330542793015, -347.1945156574853968 ) ) ;
#29651=CARTESIAN_POINT ( 'NONE',  ( -85.74333724841939386, -285.6936461556302902, -215.6184101304806688 ) ) ;
#29652=CARTESIAN_POINT ( 'NONE',  ( 102.7371733172544026, 116.6117108518458849, -282.8160689236807457 ) ) ;
#29653=CARTESIAN_POINT ( 'NONE',  ( 43.56306698794277565, 12.70319086556685129, -330.1861164527855408 ) ) ;
#29654=CARTESIAN_POINT ( 'NONE',  ( -105.6623585921115733, -259.9751593823307871, -315.4586869756183773 ) ) ;
#29655=CARTESIAN_POINT ( 'NONE',  ( -108.7621599872536819, -277.9588375987510176, -254.4381302097820026 ) ) ;
#29656=CARTESIAN_POINT ( 'NONE',  ( 13.55958273807232572, -279.7054289642043727, -217.5335106749859619 ) ) ;
#29657=CARTESIAN_POINT ( 'NONE',  ( -13.06513110315417947, -274.0258880468310849, -197.3105020519171546 ) ) ;
#29658=CARTESIAN_POINT ( 'NONE',  ( 104.6247447840909359, 114.2303491467357190, -280.5431434108185726 ) ) ;
#29659=CARTESIAN_POINT ( 'NONE',  ( -109.9838096901949456, -277.4292583091490769, -246.4924618822047648 ) ) ;
#29660=CARTESIAN_POINT ( 'NONE',  ( -101.8346370661179066, -282.0678389936044255, -307.9444638383147890 ) ) ;
#29661=CARTESIAN_POINT ( 'NONE',  ( -47.47397414952396133, -296.9393943911057931, -345.6692253503870234 ) ) ;
#29662=CARTESIAN_POINT ( 'NONE',  ( -36.21146232590110969, -292.5590134654867143, -197.2958349120321202 ) ) ;
#29663=CARTESIAN_POINT ( 'NONE',  ( -26.41801957244197396, -287.5951950692532364, -343.0893071873571785 ) ) ;
#29664=CARTESIAN_POINT ( 'NONE',  ( 53.49099207302668191, -299.6531962426988684, -193.4152503488299715 ) ) ;
#29665=CARTESIAN_POINT ( 'NONE',  ( -96.88396652854682145, -297.3085692605815211, -228.1270261086731637 ) ) ;
#29668=CARTESIAN_POINT ( 'NONE',  ( -111.0034862210051898, -280.6867964607517365, -253.5309227219060801 ) ) ;
#29669=CARTESIAN_POINT ( 'NONE',  ( -11.64763532457017980, -281.4743203664924636, -201.6485640219812012 ) ) ;
#29670=CARTESIAN_POINT ( 'NONE',  ( -99.62193874892432177, -279.7291091066461490, -313.8943913686511564 ) ) ;
#29671=CARTESIAN_POINT ( 'NONE',  ( 27.05627497650192836, -281.0852336521578536, -305.2367434235862333 ) ) ;
#29672=CARTESIAN_POINT ( 'NONE',  ( 5.596289705310259599, -273.1250789456464645, -210.4061601779694115 ) ) ;
#29675=CARTESIAN_POINT ( 'NONE',  ( 25.18952843175291889, -275.7619677009976726, -225.6843382456580684 ) ) ;
#29677=CARTESIAN_POINT ( 'NONE',  ( 25.24712700583817337, -276.9943808510390113, -229.0375246421661757 ) ) ;
#29678=CARTESIAN_POINT ( 'NONE',  ( -111.9133656767005505, -276.9168792142654638, -287.0246408058439442 ) ) ;
#29679=ORIENTED_EDGE ( 'NONE', *, *, #60782, .F. ) ;
#29681=CARTESIAN_POINT ( 'NONE',  ( 35.01319601417345240, -283.2617440155767099, -249.2631720134422153 ) ) ;
#29682=CARTESIAN_POINT ( 'NONE',  ( -60.29995964451961044, -290.9440341732312731, -200.8420003874190627 ) ) ;
#29683=CARTESIAN_POINT ( 'NONE',  ( -3.526687819948334912, -285.8353794678967006, -201.2824517417850245 ) ) ;
#29684=CARTESIAN_POINT ( 'NONE',  ( -43.03289678459244527, -281.3646855581001773, -344.2061018596274380 ) ) ;
#29685=CARTESIAN_POINT ( 'NONE',  ( -51.14608356377940623, -281.8066404029955265, -342.6959869423694727 ) ) ;
#29686=CARTESIAN_POINT ( 'NONE',  ( 16.07959904350122216, -284.8970256550888394, -218.5202172164138119 ) ) ;
#29687=CARTESIAN_POINT ( 'NONE',  ( -57.23549509702517923, -280.9947449096526952, -199.7115077534392356 ) ) ;
#29688=CARTESIAN_POINT ( 'NONE',  ( -75.39540825008494096, -271.5449969383657844, -205.6720558086690573 ) ) ;
#29689=CARTESIAN_POINT ( 'NONE',  ( -95.19567575923966274, -283.6289367563189217, -220.6900871061976090 ) ) ;
#29690=CARTESIAN_POINT ( 'NONE',  ( -39.03643339669644519, -297.0735797004466576, -345.3419724147339025 ) ) ;
#29691=CARTESIAN_POINT ( 'NONE',  ( -62.40068736496046853, -280.6593845261911042, -201.4929380460660582 ) ) ;
#29692=CARTESIAN_POINT ( 'NONE',  ( -31.06299756793917766, -288.1314472803235844, -195.4441591420193447 ) ) ;
#29693=FACE_OUTER_BOUND ( 'NONE', #32910, .T. ) ;
#29695=CARTESIAN_POINT ( 'NONE',  ( 20.19769092011089739, -294.7991740664695612, -221.3665428511745858 ) ) ;
#29696=CARTESIAN_POINT ( 'NONE',  ( -86.43307149172063930, -275.7331791087937063, -327.1312379804949160 ) ) ;
#29698=CARTESIAN_POINT ( 'NONE',  ( 24.00710202841647600, -287.3667044554251788, -316.6264753786940673 ) ) ;
#29699=CARTESIAN_POINT ( 'NONE',  ( 11.47508901242241919, -291.1420479501269938, -214.9452667130525469 ) ) ;
#29700=CARTESIAN_POINT ( 'NONE',  ( -73.09647887856914394, -276.2214312034078603, -334.5849379539266124 ) ) ;
#29701=CARTESIAN_POINT ( 'NONE',  ( -94.55055087073878894, -295.3514543126955800, -223.0337089603132483 ) ) ;
#29702=CARTESIAN_POINT ( 'NONE',  ( -33.49928954266992065, -293.4166720004045601, -196.9559029614337078 ) ) ;
#29703=CARTESIAN_POINT ( 'NONE',  ( -37.37352853689063892, -282.5519495502701943, -195.3611179825600175 ) ) ;
#29705=CARTESIAN_POINT ( 'NONE',  ( -53.16455317388895452, -293.7312148252159432, -345.0633148318088388 ) ) ;
#29706=CARTESIAN_POINT ( 'NONE',  ( 36.06810186874872670, -289.0533909609868033, -262.7821084795058937 ) ) ;
#29707=CARTESIAN_POINT ( 'NONE',  ( -99.06048478801183421, -288.1964447471899007, -314.7090962722040786 ) ) ;
#29708=CARTESIAN_POINT ( 'NONE',  ( 20.83436606291492055, -289.6072228468266303, -315.4472600817837815 ) ) ;
#29711=CARTESIAN_POINT ( 'NONE',  ( -37.25759145717675835, -289.8539069934169561, -343.5225467091082692 ) ) ;
#29713=CARTESIAN_POINT ( 'NONE',  ( 21.19556808880022913, -289.4263085862942830, -319.7716123078234318 ) ) ;
#29714=CARTESIAN_POINT ( 'NONE',  ( -96.39193230797211243, -277.2124155529683094, -223.5479052408409473 ) ) ;
#29715=CARTESIAN_POINT ( 'NONE',  ( -107.4016407626999410, -279.2946764044959309, -238.3368548032771059 ) ) ;
#29716=CARTESIAN_POINT ( 'NONE',  ( 9.192648859285828422, -282.0991723277315373, -331.6823920704227930 ) ) ;
#29717=CARTESIAN_POINT ( 'NONE',  ( 37.62803344409771000, -285.5971482527808689, -273.8783461424195593 ) ) ;
#29719=CARTESIAN_POINT ( 'NONE',  ( -93.12115690444468896, -277.3795053782364448, -221.3569160722253457 ) ) ;
#29720=CARTESIAN_POINT ( 'NONE',  ( -38.72196233910162277, -281.0693086123899889, -345.3484204329287763 ) ) ;
#29722=CARTESIAN_POINT ( 'NONE',  ( -90.85672083596389825, -276.2743181753925228, -324.8304469205484111 ) ) ;
#29723=CARTESIAN_POINT ( 'NONE',  ( -96.94090207010110305, -282.8223639851920552, -318.6459036166726264 ) ) ;
#29724=CARTESIAN_POINT ( 'NONE',  ( -107.3540425892165189, -273.6375896358426303, -248.9537119329646941 ) ) ;
#29725=CARTESIAN_POINT ( 'NONE',  ( -108.5288931497206590, -292.4066420526079355, -250.8977172977807015 ) ) ;
#29726=CARTESIAN_POINT ( 'NONE',  ( -31.96955077377693044, -299.4332532737373640, -193.8530929171411685 ) ) ;
#29727=CARTESIAN_POINT ( 'NONE',  ( 35.62283468078590687, -275.2710516445213784, -274.3180060180289388 ) ) ;
#29728=CARTESIAN_POINT ( 'NONE',  ( -97.18517654658869276, -297.9339028520907959, -315.5902180864870843 ) ) ;
#29729=CARTESIAN_POINT ( 'NONE',  ( 14.60527427079775897, -288.5118035591880243, -327.2709647863877649 ) ) ;
#29730=CARTESIAN_POINT ( 'NONE',  ( 16.21993980794121271, -278.8844712294798569, -216.9917134188006855 ) ) ;
#29731=CARTESIAN_POINT ( 'NONE',  ( -61.68656851459968493, -291.5778041804223335, -197.2547913010251364 ) ) ;
#29732=CARTESIAN_POINT ( 'NONE',  ( -50.80644922200760050, -288.2870082993838992, -342.3998316710440690 ) ) ;
#29733=CARTESIAN_POINT ( 'NONE',  ( -11.76386655225271305, -292.7191181844610242, -340.9199342683379541 ) ) ;
#29736=CARTESIAN_POINT ( 'NONE',  ( -95.00300048304677603, -289.4279681657196761, -315.2496168284164355 ) ) ;
#29738=CARTESIAN_POINT ( 'NONE',  ( -18.25216422122220905, -287.2334494808496856, -195.9529088622287816 ) ) ;
#29739=CARTESIAN_POINT ( 'NONE',  ( 30.89617123739170168, -289.8376638359844719, -254.7536222014695397 ) ) ;
#29740=CARTESIAN_POINT ( 'NONE',  ( 4.090187254265777561, -293.5676309641667103, -335.0473681626875759 ) ) ;
#29741=CARTESIAN_POINT ( 'NONE',  ( -3.098444572333995062, -283.9245090316514961, -338.7913035223452312 ) ) ;
#29742=CARTESIAN_POINT ( 'NONE',  ( -108.6644501535277669, -284.5914832033960806, -254.7443171341209904 ) ) ;
#29743=CARTESIAN_POINT ( 'NONE',  ( 32.57244656632658319, -277.1658799861546640, -293.0162624318310804 ) ) ;
#29744=CARTESIAN_POINT ( 'NONE',  ( 18.28995487035879108, -292.2687581093666154, -320.1495058370633160 ) ) ;
#29745=CARTESIAN_POINT ( 'NONE',  ( 34.22434477708029732, -274.1326527220981006, -254.0127974215033930 ) ) ;
#29747=CARTESIAN_POINT ( 'NONE',  ( 201.7194887906492795, 294.2213704821156739, -83.28174295417332473 ) ) ;
#29748=CARTESIAN_POINT ( 'NONE',  ( -4.515403015387063235, -294.2980979854356747, -340.0044460302239031 ) ) ;
#29749=CARTESIAN_POINT ( 'NONE',  ( 27.61216122733912570, -288.9832629575090550, -233.8921314275067971 ) ) ;
#29750=CARTESIAN_POINT ( 'NONE',  ( -112.8372558150556273, -297.8011794446631484, -256.8735836710407057 ) ) ;
#29751=CARTESIAN_POINT ( 'NONE',  ( 32.76537310381092993, -287.9293844090824450, -249.6072950097953367 ) ) ;
#29752=CARTESIAN_POINT ( 'NONE',  ( -67.62684590583617705, -276.4986784579949699, -340.8992648155894472 ) ) ;
#29753=CARTESIAN_POINT ( 'NONE',  ( 23.95275577669692524, -294.8230175471387611, -316.7971219267862466 ) ) ;
#29754=CARTESIAN_POINT ( 'NONE',  ( 4.849513116717326433, -286.6283170989492532, -333.2912936024492865 ) ) ;
#29755=CARTESIAN_POINT ( 'NONE',  ( -27.74626068950224322, -295.2668818956235555, -346.7928735307040711 ) ) ;
#29756=CARTESIAN_POINT ( 'NONE',  ( -94.31006874709630949, -291.5310353280050890, -224.6609182701506597 ) ) ;
#29759=CARTESIAN_POINT ( 'NONE',  ( -62.10227321113477927, -183.1506894772463170, -358.8537685376831519 ) ) ;
#29760=CARTESIAN_POINT ( 'NONE',  ( 1.155022920908411965, -288.0764393216227859, -204.4618544009913137 ) ) ;
#29761=CARTESIAN_POINT ( 'NONE',  ( -119.3990491898856732, -282.0523547857346784, -270.3284710469131937 ) ) ;
#29764=CARTESIAN_POINT ( 'NONE',  ( -92.99424422427587444, -278.6279363653633254, -217.2180408081439396 ) ) ;
#29765=CARTESIAN_POINT ( 'NONE',  ( 32.04369037306253887, -283.9184661579258204, -298.3913874970971278 ) ) ;
#29766=CARTESIAN_POINT ( 'NONE',  ( -37.67646286175954629, -140.7588499655415717, -363.8534987691544984 ) ) ;
#29768=CARTESIAN_POINT ( 'NONE',  ( -97.59110767480697746, -282.4941414840032508, -317.3570240334217942 ) ) ;
#29769=CARTESIAN_POINT ( 'NONE',  ( -2.717962632440341864, -286.6708970228537510, -336.3159260395974002 ) ) ;
#29770=CARTESIAN_POINT ( 'NONE',  ( 1.759910812504751787, -276.4297121997193472, -205.4660526705447978 ) ) ;
#29771=CARTESIAN_POINT ( 'NONE',  ( -108.5384183649809415, -297.2606848406528570, -253.9594182480530264 ) ) ;
#29772=CARTESIAN_POINT ( 'NONE',  ( -66.26252143338784606, -294.1237160610095316, -337.9246404924402896 ) ) ;
#29773=CARTESIAN_POINT ( 'NONE',  ( -79.86133719354405969, -280.1451829868925643, -206.2238955369903977 ) ) ;
#29774=CARTESIAN_POINT ( 'NONE',  ( -35.11763588454444829, -277.0234491840425335, -343.3272302418863546 ) ) ;
#29775=CARTESIAN_POINT ( 'NONE',  ( -89.54056185941973922, -278.6412010428995245, -219.1115467767951372 ) ) ;
#29776=CARTESIAN_POINT ( 'NONE',  ( -63.46477523918077424, -274.7992083076206882, -198.2564894473110826 ) ) ;
#29777=CARTESIAN_POINT ( 'NONE',  ( 10.32314135161459312, -275.3325809395210513, -330.5084956586987914 ) ) ;
#29778=CARTESIAN_POINT ( 'NONE',  ( 179.6752721477509169, 254.2973581423329961, -166.6431896920282156 ) ) ;
#29779=CARTESIAN_POINT ( 'NONE',  ( -10.71106274343912368, -274.7048202316581182, -340.5280600799721924 ) ) ;
#29780=CARTESIAN_POINT ( 'NONE',  ( -110.6449482852799946, -297.7042436808759476, -291.9766556290427388 ) ) ;
#29782=CARTESIAN_POINT ( 'NONE',  ( -101.2450674239233592, -254.4445186991787295, -323.9438275447045612 ) ) ;
#29783=CARTESIAN_POINT ( 'NONE',  ( -97.61790235991986719, -286.2109432409814076, -228.6135647561198994 ) ) ;
#29784=CARTESIAN_POINT ( 'NONE',  ( -112.5925965042998769, -286.1739043468507475, -281.2807622910634677 ) ) ;
#29785=CARTESIAN_POINT ( 'NONE',  ( -44.02544850248704478, -285.3139989042971933, -197.5653751410347070 ) ) ;
#29786=CARTESIAN_POINT ( 'NONE',  ( -93.68795063020233727, -277.6222391076884719, -222.6810054055959824 ) ) ;
#29787=CARTESIAN_POINT ( 'NONE',  ( -93.47790634488630701, -285.7317266225302888, -318.9560847290463812 ) ) ;
#29788=CARTESIAN_POINT ( 'NONE',  ( -95.32449036965496703, -277.6675213438728065, -224.8578092472863830 ) ) ;
#29789=CARTESIAN_POINT ( 'NONE',  ( -74.15666704628830530, -278.6335669687546783, -333.7557887727306252 ) ) ;
#29790=CARTESIAN_POINT ( 'NONE',  ( 24.03949023665031604, -276.5937399026541925, -310.0819035771052654 ) ) ;
#29791=CARTESIAN_POINT ( 'NONE',  ( 6.084558092747128555, -281.4280190228291758, -206.9709064587487717 ) ) ;
#29792=CARTESIAN_POINT ( 'NONE',  ( -18.92704234247923978, -283.3137170489985692, -345.1182903697914526 ) ) ;
#29794=VERTEX_POINT ( 'NONE', #38726 ) ;
#29796=CARTESIAN_POINT ( 'NONE',  ( 23.17020799508900808, -290.0295222843496390, -315.9529424533939164 ) ) ;
#29797=CARTESIAN_POINT ( 'NONE',  ( -113.7595386947123188, -289.1905403695295149, -274.0505922470043174 ) ) ;
#29798=CARTESIAN_POINT ( 'NONE',  ( -91.95864403717160940, -296.4438922646780270, -221.6826713633446957 ) ) ;
#29799=CARTESIAN_POINT ( 'NONE',  ( -58.90214686079597328, -291.1289142516320680, -196.5474341360076096 ) ) ;
#29800=CARTESIAN_POINT ( 'NONE',  ( 36.34830397062242469, -286.0411795505942791, -271.0618650333080382 ) ) ;
#29802=CARTESIAN_POINT ( 'NONE',  ( 31.77846675940804744, -289.0841707938824356, -295.0498407896378126 ) ) ;
#29803=CARTESIAN_POINT ( 'NONE',  ( -85.33152481854864391, -293.9090924074130839, -210.2361428286349110 ) ) ;
#29804=CARTESIAN_POINT ( 'NONE',  ( -3.928262803169098039, -290.6116789329420271, -337.5210523720245988 ) ) ;
#29805=CARTESIAN_POINT ( 'NONE',  ( -2.669583632924863892, -286.5945727649223613, -337.0534921139679341 ) ) ;
#29806=CARTESIAN_POINT ( 'NONE',  ( -76.24198274950093435, -284.5269780908135999, -332.4708768190238288 ) ) ;
#29807=CARTESIAN_POINT ( 'NONE',  ( -111.5460350991995568, -292.3987112919415949, -282.3504924057641006 ) ) ;
#29808=CARTESIAN_POINT ( 'NONE',  ( 82.17145489947652948, -297.7796885176689443, -194.3909460517409400 ) ) ;
#29810=CARTESIAN_POINT ( 'NONE',  ( -110.8446223043016090, -274.7442409379967216, -253.7560814164667704 ) ) ;
#29811=CARTESIAN_POINT ( 'NONE',  ( 5.678810554957125944, -281.6493811923922976, -329.5374425309335606 ) ) ;
#29812=CARTESIAN_POINT ( 'NONE',  ( -107.0828554234159782, -282.1911459966474354, -298.0919542509653297 ) ) ;
#29813=CARTESIAN_POINT ( 'NONE',  ( 37.62412235618065637, -292.9613778286965839, -287.2812034886450760 ) ) ;
#29814=CARTESIAN_POINT ( 'NONE',  ( -105.3013900511996894, -271.1821081635329733, -240.9148730300615000 ) ) ;
#29815=CARTESIAN_POINT ( 'NONE',  ( 33.88729742345162776, -273.9133530706120041, -292.0326489164241366 ) ) ;
#29816=CARTESIAN_POINT ( 'NONE',  ( -110.8680053135456518, -297.8885935144015775, -268.7386087679097955 ) ) ;
#29818=CARTESIAN_POINT ( 'NONE',  ( -92.96320937524791361, -294.0767609092507087, -322.1511459606825269 ) ) ;
#29819=CARTESIAN_POINT ( 'NONE',  ( 19.29814411840298050, -295.6384095970662997, -317.3430609234796407 ) ) ;
#29821=CARTESIAN_POINT ( 'NONE',  ( -47.80604814447011108, -295.9913262450705247, -342.8217581472771371 ) ) ;
#29822=CARTESIAN_POINT ( 'NONE',  ( 151.9709352735115147, -299.5541904835127980, -195.3611179825600175 ) ) ;
#29823=CARTESIAN_POINT ( 'NONE',  ( -106.4082784846803520, -282.9663592302003394, -240.0941494502931448 ) ) ;
#29824=CARTESIAN_POINT ( 'NONE',  ( -109.2758583226734999, -296.7161096486238421, -257.9322449509696753 ) ) ;
#29825=CARTESIAN_POINT ( 'NONE',  ( -105.4320937364439459, -285.0176559456355676, -234.2928403639612043 ) ) ;
#29826=CARTESIAN_POINT ( 'NONE',  ( 31.09865369464192497, -283.8915037598907816, -302.5037184260195318 ) ) ;
#29827=CARTESIAN_POINT ( 'NONE',  ( 14.58631384061667902, -288.0119228364881678, -327.2596236029493184 ) ) ;
#29828=CARTESIAN_POINT ( 'NONE',  ( -25.08432277463506921, -290.2085090175638129, -196.4856837645282326 ) ) ;
#29829=CARTESIAN_POINT ( 'NONE',  ( -112.5573669640215400, -277.9469855783382854, -254.5890389006116266 ) ) ;
#29830=CARTESIAN_POINT ( 'NONE',  ( -85.33152481854862970, -281.1952119285918457, -330.4860931364851808 ) ) ;
#29832=CARTESIAN_POINT ( 'NONE',  ( 34.10033695288255018, -286.1255794015199854, -253.4792213777357688 ) ) ;
#29833=CARTESIAN_POINT ( 'NONE',  ( -110.9316640555430951, -289.7443468063224259, -248.7738597223181785 ) ) ;
#29834=DIRECTION ( 'NONE',  ( 0.000000000000000000, 0.000000000000000000, 1.000000000000000000 ) ) ;
#29835=CARTESIAN_POINT ( 'NONE',  ( -104.4545002634570778, -298.5632294854839870, -239.5409319625470062 ) ) ;
#29836=CARTESIAN_POINT ( 'NONE',  ( -104.2861592644941169, -280.4582188159449174, -233.5230170216956935 ) ) ;
#29837=CARTESIAN_POINT ( 'NONE',  ( -27.97776951857643013, -292.9540812017858684, -345.1844125850856244 ) ) ;
#29838=CARTESIAN_POINT ( 'NONE',  ( 27.80217441984163429, -280.7697317689558076, -237.2586403522886087 ) ) ;
#29839=CARTESIAN_POINT ( 'NONE',  ( 25.71587312414331805, -294.3034169401998952, -314.5739754410757882 ) ) ;
#29840=CARTESIAN_POINT ( 'NONE',  ( -4.100380887461235524, -284.5668441562411317, -202.4916536080753815 ) ) ;
#29841=CARTESIAN_POINT ( 'NONE',  ( -109.5089367781370555, -280.2895844519035791, -290.7790171108649133 ) ) ;
#29842=CARTESIAN_POINT ( 'NONE',  ( -88.67529979404858409, -294.8526760979827372, -322.6652419775610952 ) ) ;
#29845=CARTESIAN_POINT ( 'NONE',  ( 34.69441767856497449, -283.2787612697925965, -250.7509760322479906 ) ) ;
#29846=CARTESIAN_POINT ( 'NONE',  ( -42.40023858212408925, -294.6253196379149131, -343.2473281353082371 ) ) ;
#29848=CARTESIAN_POINT ( 'NONE',  ( -69.91165696735023971, -274.9809262143061233, -337.9199732462171255 ) ) ;
#29849=CARTESIAN_POINT ( 'NONE',  ( -44.01851614842487947, -273.1670796337138540, -193.7600351154993348 ) ) ;
#29851=CARTESIAN_POINT ( 'NONE',  ( -99.71050631250705010, -290.9079440987432008, -232.4252244301009114 ) ) ;
#29852=CARTESIAN_POINT ( 'NONE',  ( -39.74303679590553884, -281.5416073825505237, -196.6942784055590039 ) ) ;
#29853=CARTESIAN_POINT ( 'NONE',  ( 19.60328686438878520, -276.4941641392466636, -223.4174403061531962 ) ) ;
#29854=CARTESIAN_POINT ( 'NONE',  ( -37.29407993814776034, -284.6516504174961710, -346.5740357033037071 ) ) ;
#29855=CARTESIAN_POINT ( 'NONE',  ( 28.50052263533785180, -280.7855805256578492, -302.9099147549125632 ) ) ;
#29856=CARTESIAN_POINT ( 'NONE',  ( -79.74225785221808849, -279.6250536594727123, -332.2886568374822787 ) ) ;
#29858=CARTESIAN_POINT ( 'NONE',  ( -55.33155968404423675, -273.6601949049922382, -195.4921326973236262 ) ) ;
#29859=CARTESIAN_POINT ( 'NONE',  ( 22.95707219933349563, -294.8731732784926862, -226.6888813508244027 ) ) ;
#29862=CARTESIAN_POINT ( 'NONE',  ( 32.27213237797947443, -292.0803596796338866, -300.3970232711724861 ) ) ;
#29863=CARTESIAN_POINT ( 'NONE',  ( -4.071069848576229333, -274.0108493904762099, -205.3005232761462935 ) ) ;
#29865=CARTESIAN_POINT ( 'NONE',  ( 23.41136716800506079, -294.4511363629974312, -224.1685001544242937 ) ) ;
#29866=CARTESIAN_POINT ( 'NONE',  ( -114.2704648735229114, -281.0519495502701943, -270.3937649182068981 ) ) ;
#29867=CARTESIAN_POINT ( 'NONE',  ( -70.73853485298552357, -292.8264709683612068, -201.4215781596171269 ) ) ;
#29869=CARTESIAN_POINT ( 'NONE',  ( -48.30502295628507170, -291.1920234105690497, -344.4393204964492270 ) ) ;
#29870=CARTESIAN_POINT ( 'NONE',  ( 37.53276211602584311, -273.5684581208294048, -271.6411216969615907 ) ) ;
#29871=CARTESIAN_POINT ( 'NONE',  ( -21.31971061796216205, -278.7653718859305059, -343.1094634837012336 ) ) ;
#29872=CARTESIAN_POINT ( 'NONE',  ( -6.184020329435577779, -292.7193597693570268, -337.9666886910082439 ) ) ;
#29873=CARTESIAN_POINT ( 'NONE',  ( -39.57497621063551918, -281.8848327648923373, -194.6163948914206401 ) ) ;
#29875=CARTESIAN_POINT ( 'NONE',  ( -16.13041171608157853, -282.4369113983623834, -340.2336356887971078 ) ) ;
#29876=CARTESIAN_POINT ( 'NONE',  ( -82.06976748427655366, -280.5375797162723757, -208.0643082766190730 ) ) ;
#29877=CARTESIAN_POINT ( 'NONE',  ( 4.316821878109750266, -281.2991373976518048, -334.7089206967824566 ) ) ;
#29878=CARTESIAN_POINT ( 'NONE',  ( -80.08519197534438661, -278.5562526798925091, -334.1888374775280681 ) ) ;
#29880=CARTESIAN_POINT ( 'NONE',  ( -5.555776691504733300, -278.1617103164889500, -339.7323139232078120 ) ) ;
#29882=CARTESIAN_POINT ( 'NONE',  ( -37.30987171927208124, -285.5519495502701375, -340.3611179825599606 ) ) ;
#29884=CARTESIAN_POINT ( 'NONE',  ( -37.16992363897267637, -300.0544674696619722, -195.3581240247519588 ) ) ;
#29885=CARTESIAN_POINT ( 'NONE',  ( -26.81390449538187681, -274.9376996216893190, -344.2597804861110831 ) ) ;
#29886=CARTESIAN_POINT ( 'NONE',  ( -81.36182585714203697, -293.2226735973649738, -208.4240326264954035 ) ) ;
#29887=CARTESIAN_POINT ( 'NONE',  ( -14.80711000723318271, -291.7005820484347396, -200.8191528386145137 ) ) ;
#29888=CARTESIAN_POINT ( 'NONE',  ( 5.517839968940424278, -287.9961654821806860, -334.2562408463186898 ) ) ;
#29890=CARTESIAN_POINT ( 'NONE',  ( 32.79082963577867815, -291.7373925767483911, -240.0290465019735962 ) ) ;
#29891=CARTESIAN_POINT ( 'NONE',  ( -87.48720168815138720, -282.1653598646322507, -324.5777872468449914 ) ) ;
#29892=CARTESIAN_POINT ( 'NONE',  ( -110.8426426442360366, -292.2762838640759355, -280.8673370803383023 ) ) ;
#29893=CARTESIAN_POINT ( 'NONE',  ( -108.0143939209926316, -283.3078378712709195, -249.3018142383234874 ) ) ;
#29894=CARTESIAN_POINT ( 'NONE',  ( 10.24064517707352628, -283.6951550247052865, -326.4384471757738311 ) ) ;
#29895=CARTESIAN_POINT ( 'NONE',  ( -12.28915658069333894, -289.6754272798460761, -342.9784532819220999 ) ) ;
#29896=CARTESIAN_POINT ( 'NONE',  ( 35.62769696183987378, -282.0928510664701889, -274.0292959800119661 ) ) ;
#29897=CARTESIAN_POINT ( 'NONE',  ( 32.96606803641201822, -291.9575536951258528, -239.9501585557781596 ) ) ;
#29898=CARTESIAN_POINT ( 'NONE',  ( -7.415474350190210728, -287.2373957677201588, -199.5332645620786991 ) ) ;
#29899=CARTESIAN_POINT ( 'NONE',  ( 37.08647723653804462, -288.2886935976654854, -289.8540222710630019 ) ) ;
#29900=CARTESIAN_POINT ( 'NONE',  ( -103.4863637256166840, -285.1373171418991888, -239.3562761901939098 ) ) ;
#29903=CARTESIAN_POINT ( 'NONE',  ( -8.830514221867677094, -296.5436719518422706, -340.6122701827032415 ) ) ;
#29904=CARTESIAN_POINT ( 'NONE',  ( -61.45214101821655817, -294.0436133027067171, -343.0249402414153792 ) ) ;
#29905=CARTESIAN_POINT ( 'NONE',  ( -109.3613197716933172, -277.7856305141615962, -257.0726705564470080 ) ) ;
#29906=CARTESIAN_POINT ( 'NONE',  ( -9.148401514218059916, -297.7450392380144990, -193.4660680483073634 ) ) ;
#29907=CARTESIAN_POINT ( 'NONE',  ( 34.74175376992908326, -292.2330047438293263, -285.7409537183996804 ) ) ;
#29908=CARTESIAN_POINT ( 'NONE',  ( -3.663327443979457421, -276.2629734623603213, -204.4398270365678627 ) ) ;
#29909=CARTESIAN_POINT ( 'NONE',  ( -107.8412844219014914, -294.4953213123518481, -293.0612262769406584 ) ) ;
#29910=CARTESIAN_POINT ( 'NONE',  ( 26.14376430493017978, -295.2598141657338147, -307.1948838743196575 ) ) ;
#29911=CARTESIAN_POINT ( 'NONE',  ( 19.07977054083941226, -295.2928646163152280, -317.1675675605621336 ) ) ;
#29913=CARTESIAN_POINT ( 'NONE',  ( 3.216127482886622424, -292.5088930857937726, -333.7081762068345370 ) ) ;
#29914=CARTESIAN_POINT ( 'NONE',  ( -38.50419039950298838, -300.0377411448425278, -195.3669752758073059 ) ) ;
#29915=CARTESIAN_POINT ( 'NONE',  ( -110.0215577713507002, -291.3750310829137788, -279.3637143287406843 ) ) ;
#29916=CARTESIAN_POINT ( 'NONE',  ( -10.47827546018375955, -295.0250189982331221, -338.2613676279515289 ) ) ;
#29917=CARTESIAN_POINT ( 'NONE',  ( -109.0926182891334690, -280.2342611680612663, -293.5552870345799192 ) ) ;
#29918=CARTESIAN_POINT ( 'NONE',  ( -56.41740065600621534, -278.4962791015083212, -196.2158807661456876 ) ) ;
#29919=EDGE_LOOP ( 'NONE', ( #29679, #82295, #69915, #56670 ) ) ;
#29920=CARTESIAN_POINT ( 'NONE',  ( 30.44928143128743159, -275.3718034325327721, -306.7736058058741264 ) ) ;
#29921=CARTESIAN_POINT ( 'NONE',  ( 26.78739038945298034, -280.1423610684755090, -308.2620461847151887 ) ) ;
#29922=CARTESIAN_POINT ( 'NONE',  ( -61.77165505891698416, -278.1398734266709880, -198.1277936867041376 ) ) ;
#29923=CARTESIAN_POINT ( 'NONE',  ( -81.14922814223729119, -277.4582436486327879, -209.2797876668647348 ) ) ;
#29924=CARTESIAN_POINT ( 'NONE',  ( -90.39030626128513290, -295.9667943502856247, -219.4248735958797454 ) ) ;
#29925=CARTESIAN_POINT ( 'NONE',  ( 29.54807319997954451, -278.0019850777950978, -304.3971766632907361 ) ) ;
#29927=CARTESIAN_POINT ( 'NONE',  ( -97.02963520811226772, -289.1997129887546976, -224.3428877661676495 ) ) ;
#29928=CARTESIAN_POINT ( 'NONE',  ( -96.39105601114142985, -289.8868828867213097, -319.7999217175851641 ) ) ;
#29929=CARTESIAN_POINT ( 'NONE',  ( 22.99271303944037825, -276.9416516797861618, -225.5304697936171010 ) ) ;
#29930=CARTESIAN_POINT ( 'NONE',  ( -34.36391085241772458, -296.0893536768662102, -195.5287939806827637 ) ) ;
#29931=CARTESIAN_POINT ( 'NONE',  ( -108.8744024482532637, -284.1073652428066225, -242.1588253247516320 ) ) ;
#29933=CARTESIAN_POINT ( 'NONE',  ( -20.12043501171388016, -280.8308371697673351, -343.4099304285018093 ) ) ;
#29935=CARTESIAN_POINT ( 'NONE',  ( 19.66384094117455561, -291.6963196589528025, -224.1081426606676530 ) ) ;
#29936=CARTESIAN_POINT ( 'NONE',  ( -77.70106369195956120, -283.6439682641382092, -207.9945426840557730 ) ) ;
#29939=CARTESIAN_POINT ( 'NONE',  ( -14.20589505014096865, -290.3520520576256558, -199.0187380789768952 ) ) ;
#29940=CARTESIAN_POINT ( 'NONE',  ( -45.98175064150800040, -278.7635263870486710, -343.7047937132116431 ) ) ;
#29941=CARTESIAN_POINT ( 'NONE',  ( -4.321026238989570167, -283.8316289799137166, -339.4960361997546556 ) ) ;
#29942=CARTESIAN_POINT ( 'NONE',  ( 18.97918180914302155, -272.9351792204907952, -219.9128512809309086 ) ) ;
#29943=CARTESIAN_POINT ( 'NONE',  ( -74.72010898547075897, -285.5395231114922581, -207.6566161402693638 ) ) ;
#29944=CARTESIAN_POINT ( 'NONE',  ( 31.66460719816356573, -276.6392655624655958, -244.7973845798202319 ) ) ;
#29945=CARTESIAN_POINT ( 'NONE',  ( -26.98858078803188221, -277.7199761807559639, -342.7863528566958280 ) ) ;
#29946=CARTESIAN_POINT ( 'NONE',  ( -112.2100460062138154, -286.4849981602699245, -275.6040226308801948 ) ) ;
#29950=CARTESIAN_POINT ( 'NONE',  ( -101.6294381441484944, -295.8271253558790477, -312.8378140282363233 ) ) ;
#29951=CARTESIAN_POINT ( 'NONE',  ( 35.59798520561974300, -289.3273886906071084, -254.4976659571739219 ) ) ;
#29953=CARTESIAN_POINT ( 'NONE',  ( -99.90806341382572953, -275.6948066931273047, -220.5068182859052968 ) ) ;
#29954=CARTESIAN_POINT ( 'NONE',  ( -112.0973290108608609, -277.6874567816421404, -253.2412914115491560 ) ) ;
#29955=CARTESIAN_POINT ( 'NONE',  ( -79.13840184732436001, -289.8987236365313152, -206.5840362964534336 ) ) ;
#29956=CARTESIAN_POINT ( 'NONE',  ( -25.04500570273807014, -287.7317941831717576, -197.6491729531099679 ) ) ;
#29957=CARTESIAN_POINT ( 'NONE',  ( -109.4687845484847060, -280.0955420808243161, -287.0201548553062025 ) ) ;
#29958=CARTESIAN_POINT ( 'NONE',  ( 37.53455404474896540, -289.1694423256822688, -285.5976811034396405 ) ) ;
#29959=CARTESIAN_POINT ( 'NONE',  ( -48.60455954803998679, -285.1957341592250259, -344.5106199646174332 ) ) ;
#29960=CARTESIAN_POINT ( 'NONE',  ( -97.05304629950505557, -278.0662367969564457, -318.9981729088901261 ) ) ;
#29961=CARTESIAN_POINT ( 'NONE',  ( -110.3172003782366062, -270.7652409192697291, -253.7899142056186292 ) ) ;
#29962=CARTESIAN_POINT ( 'NONE',  ( -112.9957817693692732, -278.5656195732849483, -255.9567391137153152 ) ) ;
#29963=CARTESIAN_POINT ( 'NONE',  ( -111.5769001271281269, -274.4122687124617528, -270.3847510867740311 ) ) ;
#29966=CARTESIAN_POINT ( 'NONE',  ( 21.31550574532285580, -290.6948066931273615, -317.0979686699210447 ) ) ;
#29967=CARTESIAN_POINT ( 'NONE',  ( -27.11047220429551174, -272.4202254892947508, -195.0136625216094615 ) ) ;
#29969=CARTESIAN_POINT ( 'NONE',  ( -96.45180268998970519, -278.6602774360619605, -227.4194806487598157 ) ) ;
#29970=CARTESIAN_POINT ( 'NONE',  ( 38.09837004603772215, -276.5891256373307669, -256.9894630542547134 ) ) ;
#29971=CARTESIAN_POINT ( 'NONE',  ( -58.08813825178550161, -299.2040577398817049, -199.7568672537821044 ) ) ;
#29972=CARTESIAN_POINT ( 'NONE',  ( -41.56820766288251434, -282.1627741289096889, -347.0615513430716419 ) ) ;
#29973=CARTESIAN_POINT ( 'NONE',  ( 35.76360814735154747, -289.4637323633321557, -282.0000611686700722 ) ) ;
#29974=CARTESIAN_POINT ( 'NONE',  ( -67.91758684803448887, -299.1782786398678127, -200.3918572842549963 ) ) ;
#29975=CARTESIAN_POINT ( 'NONE',  ( -30.54390017808885105, -299.3405499070659062, -193.7568310456069014 ) ) ;
#29976=CARTESIAN_POINT ( 'NONE',  ( -31.43280527507423017, -296.9776604949606167, -345.0121771037880762 ) ) ;
#29977=CARTESIAN_POINT ( 'NONE',  ( 21.12393328062062636, -278.9083044070519009, -223.6513958520252743 ) ) ;
#29978=CARTESIAN_POINT ( 'NONE',  ( -29.79914699245145471, -272.1682200242870522, -196.0983635609978819 ) ) ;
#29979=CARTESIAN_POINT ( 'NONE',  ( -12.97897202332027433, -287.9636950450033623, -198.1607170584861706 ) ) ;
#29980=CARTESIAN_POINT ( 'NONE',  ( -56.15814081689888582, -288.2204752797404694, -341.2670414578177542 ) ) ;
#29981=CARTESIAN_POINT ( 'NONE',  ( 186.8782473919017946, 262.4247097882764592, -153.1099460133960974 ) ) ;
#29983=CARTESIAN_POINT ( 'NONE',  ( -15.14092496997311876, -287.3450151944473419, -343.5309504060106178 ) ) ;
#29984=CARTESIAN_POINT ( 'NONE',  ( -71.18632843777302810, -289.1785425819629722, -335.0794072839310047 ) ) ;
#29986=CARTESIAN_POINT ( 'NONE',  ( -99.10351695446293263, -286.2392355891583975, -224.8097733468155184 ) ) ;
#29987=CARTESIAN_POINT ( 'NONE',  ( -51.28076609988519152, -277.5685932409912766, -342.0394963578903003 ) ) ;
#29989=CARTESIAN_POINT ( 'NONE',  ( 30.62203016183847382, -292.9327422715573448, -305.8917227337423128 ) ) ;
#29990=CARTESIAN_POINT ( 'NONE',  ( 9.153773371139244830, -283.0837082272484508, -331.6104749617016978 ) ) ;
#29991=CARTESIAN_POINT ( 'NONE',  ( 20.52753454325547366, -282.3945893470113333, -220.6033485129433700 ) ) ;
#29992=CARTESIAN_POINT ( 'NONE',  ( -92.41564587003446718, -284.1474507654099853, -324.1440594408492188 ) ) ;
#29993=CARTESIAN_POINT ( 'NONE',  ( 31.08863166773339515, -281.5439148762067134, -244.7331965685933142 ) ) ;
#29994=CARTESIAN_POINT ( 'NONE',  ( -39.40415736724759910, -139.7686915660002001, -364.8644887815387392 ) ) ;
#29995=CARTESIAN_POINT ( 'NONE',  ( -97.55334013989948971, -279.9444796973232314, -314.8189110281763874 ) ) ;
#29996=CARTESIAN_POINT ( 'NONE',  ( -78.88083861134452945, -207.7982064915168223, -356.3615181246614725 ) ) ;
#29997=CARTESIAN_POINT ( 'NONE',  ( -112.4673293132808567, -270.3863210923503289, -283.6829518252387743 ) ) ;
#29998=CARTESIAN_POINT ( 'NONE',  ( -109.7410405708451862, -271.8925054879165373, -259.4825570268374690 ) ) ;
#29999=CARTESIAN_POINT ( 'NONE',  ( 33.35754084228669569, -293.4482082417355286, -300.8459974687801832 ) ) ;
#30000=CARTESIAN_POINT ( 'NONE',  ( 139.4533679669662263, 178.0281513006911212, -238.5041391399041402 ) ) ;
#30001=CARTESIAN_POINT ( 'NONE',  ( 13.64836042249343784, -273.4334447296446342, -213.2524958372876824 ) ) ;
#30002=CARTESIAN_POINT ( 'NONE',  ( -72.76051505210691062, -287.9294662818647339, -335.1063723694215923 ) ) ;
#30003=CARTESIAN_POINT ( 'NONE',  ( -56.09280974463298008, -297.1565140623127945, -342.2423811376186222 ) ) ;
#30004=CARTESIAN_POINT ( 'NONE',  ( -34.54255373928891260, -290.3315618426191804, -343.8508612348118163 ) ) ;
#30006=CARTESIAN_POINT ( 'NONE',  ( -98.08091297443648671, -296.8648691639485264, -317.3032977012418883 ) ) ;
#30007=CARTESIAN_POINT ( 'NONE',  ( -67.57888449906954520, -286.1367378164160300, -203.8502081770367340 ) ) ;
#30008=CARTESIAN_POINT ( 'NONE',  ( 75.67381866370362786, -298.2323840635743295, -193.7806729451839942 ) ) ;
#30009=CARTESIAN_POINT ( 'NONE',  ( -33.55756416519896845, -292.9014776589032181, -193.6158305978021588 ) ) ;
#30010=CARTESIAN_POINT ( 'NONE',  ( 38.54662636682888177, -294.2040597308703127, -283.1094011584139594 ) ) ;
#30012=CARTESIAN_POINT ( 'NONE',  ( -33.51055871306127187, -292.2683635459865172, -197.4492268861841069 ) ) ;
#30014=CARTESIAN_POINT ( 'NONE',  ( -108.7491497465764496, -274.7896804215772590, -245.6570629309408105 ) ) ;
#30015=CARTESIAN_POINT ( 'NONE',  ( 35.67946665432231157, -274.6395634983861669, -293.5110190674261617 ) ) ;
#30017=CARTESIAN_POINT ( 'NONE',  ( -70.28036672877185254, -276.9822713270783083, -339.9066247533874616 ) ) ;
#30019=CARTESIAN_POINT ( 'NONE',  ( -74.66052174613601267, -271.9469144356937136, -206.6328940859135059 ) ) ;
#30020=CARTESIAN_POINT ( 'NONE',  ( 20.97838420434981899, -274.3291137859762330, -316.3123259680433534 ) ) ;
#30021=CARTESIAN_POINT ( 'NONE',  ( -110.6513237473105562, -273.6675820552150640, -267.6394394776495460 ) ) ;
#30022=CARTESIAN_POINT ( 'NONE',  ( -108.1707341681382246, -273.7407859269225696, -251.5478278179002984 ) ) ;
#30023=CARTESIAN_POINT ( 'NONE',  ( -110.0738327710919719, -274.5941884866206237, -248.1808289681541453 ) ) ;
#30024=CARTESIAN_POINT ( 'NONE',  ( -8.537194773463797404, -274.6971543346402314, -340.0077547523985118 ) ) ;
#30025=CARTESIAN_POINT ( 'NONE',  ( -96.48600631320077525, -296.6028735124316995, -313.3457638829561347 ) ) ;
#30026=CARTESIAN_POINT ( 'NONE',  ( 34.89937600890105784, -292.3103621829958456, -284.3825956873396308 ) ) ;
#30028=CARTESIAN_POINT ( 'NONE',  ( -9.228462278270455954, -277.1866261001693488, -341.9793611950705667 ) ) ;
#30029=CARTESIAN_POINT ( 'NONE',  ( 32.85943054869840552, -275.4519780082069360, -250.1604922053381586 ) ) ;
#30031=CARTESIAN_POINT ( 'NONE',  ( -113.8475389179158554, -283.2419334603202969, -269.9675414550841879 ) ) ;
#30032=CARTESIAN_POINT ( 'NONE',  ( -68.73837105258257907, -297.4640084042130184, -338.6707206451707748 ) ) ;
#30035=CARTESIAN_POINT ( 'NONE',  ( -4.512958728645550366, -285.6934359570981883, -204.9785861745966713 ) ) ;
#30036=CARTESIAN_POINT ( 'NONE',  ( -89.81991322911061104, -276.0447080517561744, -322.6259787593550072 ) ) ;
#30037=CARTESIAN_POINT ( 'NONE',  ( -110.8696145703247851, -277.0875692513499189, -273.3645682251929543 ) ) ;
#30038=CARTESIAN_POINT ( 'NONE',  ( -104.0484609425845832, -286.0974965998791504, -304.7544469944687080 ) ) ;
#30039=CARTESIAN_POINT ( 'NONE',  ( -11.36396509403575550, -275.6032351762364101, -201.6606773979221430 ) ) ;
#30041=CARTESIAN_POINT ( 'NONE',  ( 25.39650288484879326, -274.5300512640397983, -313.7000507973789922 ) ) ;
#30042=CARTESIAN_POINT ( 'NONE',  ( -35.40931205529849990, -282.0764801125492340, -195.2064657382867097 ) ) ;
#30044=CARTESIAN_POINT ( 'NONE',  ( 31.39176801577343312, -289.0619864328721178, -238.8501517250077200 ) ) ;
#30046=CARTESIAN_POINT ( 'NONE',  ( 28.50831549217935290, -291.0737347051569941, -234.3548185962341677 ) ) ;
#30047=CARTESIAN_POINT ( 'NONE',  ( 82.16780035446942065, -298.0667158113331539, -196.7127616594630979 ) ) ;
#30048=CARTESIAN_POINT ( 'NONE',  ( -37.13315689824700883, -296.8497504458034655, -196.9612216088964090 ) ) ;
#30049=CARTESIAN_POINT ( 'NONE',  ( -97.75296974734445143, -289.2855391032036891, -227.1309089878609768 ) ) ;
#30050=CARTESIAN_POINT ( 'NONE',  ( -90.99921415893403775, -226.8295888252787904, -341.9546587472784154 ) ) ;
#30051=CARTESIAN_POINT ( 'NONE',  ( -37.11877477909561662, -296.0547944529405981, -195.3582583741226131 ) ) ;
#30052=CARTESIAN_POINT ( 'NONE',  ( 36.02998097164891789, -285.7647676252742599, -249.2137420695398760 ) ) ;
#30053=CARTESIAN_POINT ( 'NONE',  ( -112.4819032575698117, -282.9397404332834753, -258.7044807618646587 ) ) ;
#30054=CARTESIAN_POINT ( 'NONE',  ( -80.96091704444086190, -285.0824722826523043, -329.6928690095891170 ) ) ;
#30055=CARTESIAN_POINT ( 'NONE',  ( -32.12400417514923845, -283.7874863284671960, -343.3363012714660272 ) ) ;
#30056=CARTESIAN_POINT ( 'NONE',  ( -94.20030341461031753, -291.8489665307449741, -319.8131759508264622 ) ) ;
#30057=CARTESIAN_POINT ( 'NONE',  ( 16.00932649370802352, -275.1172660779564580, -214.8686657942969020 ) ) ;
#30058=CARTESIAN_POINT ( 'NONE',  ( -2.487126102765745195, -286.6745662429819390, -337.4019478571352124 ) ) ;
#30059=CARTESIAN_POINT ( 'NONE',  ( 20.03586956164628674, -274.8550232325782758, -218.9328398031620964 ) ) ;
#30060=CARTESIAN_POINT ( 'NONE',  ( 30.21667873787950498, -295.1112435826379397, -238.4947318829150618 ) ) ;
#30062=CARTESIAN_POINT ( 'NONE',  ( 31.98288692825981272, -290.4805209788416391, -303.7098442033569654 ) ) ;
#30063=CARTESIAN_POINT ( 'NONE',  ( -33.48699578476516336, -281.6874736373272867, -343.7657692059435135 ) ) ;
#30064=CARTESIAN_POINT ( 'NONE',  ( -110.0604580777789891, -276.3074393655558083, -289.4383380576616673 ) ) ;
#30065=CARTESIAN_POINT ( 'NONE',  ( -113.6476476313650039, -271.0681364600990264, -267.5001605809566172 ) ) ;
#30066=CARTESIAN_POINT ( 'NONE',  ( 17.50622294442265314, -275.5900778153945794, -318.7080247415787539 ) ) ;
#30067=CARTESIAN_POINT ( 'NONE',  ( 34.89229081766575291, -294.8815809324760266, -255.7680269389747139 ) ) ;
#30068=CARTESIAN_POINT ( 'NONE',  ( -3.538274810502163081, -293.4511511784415916, -205.3939194473625207 ) ) ;
#30069=CARTESIAN_POINT ( 'NONE',  ( -107.4999556749206420, -286.6230525061420735, -246.6252257697056791 ) ) ;
#30070=CARTESIAN_POINT ( 'NONE',  ( 38.63817475728407658, -294.8691996773992514, -261.7739678749244376 ) ) ;
#30071=CARTESIAN_POINT ( 'NONE',  ( 36.22532197238260920, -294.6017784424034858, -249.3088597534250539 ) ) ;
#30072=CARTESIAN_POINT ( 'NONE',  ( -95.60561350151522220, -295.7674127605293393, -314.3625748173021748 ) ) ;
#30073=CARTESIAN_POINT ( 'NONE',  ( -98.16607978952185931, -291.9549833876038178, -314.2404467087722537 ) ) ;
#30074=CARTESIAN_POINT ( 'NONE',  ( -31.63417057372542374, -283.1486881293692477, -347.1625628321319255 ) ) ;
#30075=CARTESIAN_POINT ( 'NONE',  ( -105.7181357150988390, -271.1169341839197386, -237.7272623386999442 ) ) ;
#30076=CARTESIAN_POINT ( 'NONE',  ( -111.7206598785377736, -284.6371440577562453, -250.2416453859408421 ) ) ;
#30077=CARTESIAN_POINT ( 'NONE',  ( -40.55182215883634456, -279.0725820021370964, -344.9496096060988748 ) ) ;
#30079=CARTESIAN_POINT ( 'NONE',  ( -109.5811216921551647, -283.5183593570602625, -257.3060235623159429 ) ) ;
#30081=CARTESIAN_POINT ( 'NONE',  ( 20.83714860548262848, -286.2041736574634569, -317.7123064628988800 ) ) ;
#30082=CARTESIAN_POINT ( 'NONE',  ( -102.3395509548886793, -277.2088415202943565, -231.3286469396649068 ) ) ;
#30083=CARTESIAN_POINT ( 'NONE',  ( 20.69763459394507876, -20.92298310053570987, -343.0354172471594438 ) ) ;
#30084=CARTESIAN_POINT ( 'NONE',  ( -62.57824881752455326, -285.2224795249605904, -201.7425614640241918 ) ) ;
#30085=CARTESIAN_POINT ( 'NONE',  ( -3.845167379837290955, -281.6892877888157045, -201.4555229861685746 ) ) ;
#30086=CARTESIAN_POINT ( 'NONE',  ( -103.6014096522708456, -289.1036897349030710, -309.2280077320278338 ) ) ;
#30087=CARTESIAN_POINT ( 'NONE',  ( -41.32206616372621966, -278.7015733503956767, -346.4701626419461604 ) ) ;
#30088=CARTESIAN_POINT ( 'NONE',  ( -54.00740367314978130, -278.5768304575398702, -345.0850289331229988 ) ) ;
#30089=CARTESIAN_POINT ( 'NONE',  ( -79.05312907520827537, -279.3051648116177148, -210.4515469635940690 ) ) ;
#30090=CARTESIAN_POINT ( 'NONE',  ( -5.857653699906765432, -276.4480281633591403, -202.6809759385448331 ) ) ;
#30091=CARTESIAN_POINT ( 'NONE',  ( 39.23706863851335669, -293.6588784897912205, -278.8948681107987113 ) ) ;
#30092=CARTESIAN_POINT ( 'NONE',  ( -12.76968975586291144, -286.7512578224150843, -340.8456064029622894 ) ) ;
#30093=CARTESIAN_POINT ( 'NONE',  ( 6.024049977756507523, -294.2299127158751730, -207.7044971708718037 ) ) ;
#30094=CARTESIAN_POINT ( 'NONE',  ( 3.979331734179064828, -293.4011930418107568, -330.9152127969904313 ) ) ;
#30095=CARTESIAN_POINT ( 'NONE',  ( -9.226661275993837563, -294.3409088006461616, -337.7663594828489977 ) ) ;
#30096=CARTESIAN_POINT ( 'NONE',  ( -96.34987631706967193, -292.2933245109340987, -221.3558453921922080 ) ) ;
#30097=CARTESIAN_POINT ( 'NONE',  ( 26.94863035827613373, -282.6776424858046539, -305.1554576634643468 ) ) ;
#30100=CARTESIAN_POINT ( 'NONE',  ( -110.8084256622462220, -271.8932312149723884, -247.9205677568280350 ) ) ;
#30101=CARTESIAN_POINT ( 'NONE',  ( 34.97944124457312398, -288.5357862830449562, -296.6496934112837494 ) ) ;
#30102=CARTESIAN_POINT ( 'NONE',  ( 3.853887760259127937, -280.6439027716538135, -334.0095040467646186 ) ) ;
#30103=CARTESIAN_POINT ( 'NONE',  ( -54.49277334157021357, -289.5998441888542629, -345.4597011814711323 ) ) ;
#30104=CARTESIAN_POINT ( 'NONE',  ( -39.97893106012885767, -286.3513873727571308, -197.3876125175493712 ) ) ;
#30106=CARTESIAN_POINT ( 'NONE',  ( 43.52240465396816660, 12.61540204620569661, -329.8876815671075065 ) ) ;
#30107=CARTESIAN_POINT ( 'NONE',  ( -76.97335133370192750, -207.9390729104919444, -353.3932181474779668 ) ) ;
#30108=CARTESIAN_POINT ( 'NONE',  ( -104.4235273460602116, -277.3560603860048559, -299.6879357763577900 ) ) ;
#30109=CARTESIAN_POINT ( 'NONE',  ( -83.21083283242153072, -276.6175152124334886, -327.6125498659733921 ) ) ;
#30110=CARTESIAN_POINT ( 'NONE',  ( -76.41832785919542914, -273.2116073542446202, -203.9763683654935846 ) ) ;
#30111=CARTESIAN_POINT ( 'NONE',  ( 194.7859659566919106, 275.7971500590870733, -124.4546405686035797 ) ) ;
#30112=CARTESIAN_POINT ( 'NONE',  ( -79.56991505802331233, -278.0688319646793047, -206.6157588735346451 ) ) ;
#30113=CARTESIAN_POINT ( 'NONE',  ( 6.053921781341184527, -296.2328380008998465, -332.8014734866216600 ) ) ;
#30114=CARTESIAN_POINT ( 'NONE',  ( -70.25404820465854527, -292.0985273036471881, -205.1325522621764605 ) ) ;
#30115=CARTESIAN_POINT ( 'NONE',  ( -7.792268875157949637, -275.3711503760661685, -199.4552005377946102 ) ) ;
#30116=CARTESIAN_POINT ( 'NONE',  ( -94.49831384166250814, -288.5879388392519331, -316.5603061620244603 ) ) ;
#30117=CARTESIAN_POINT ( 'NONE',  ( -71.36517467702078932, -274.2660347085600847, -201.3994187086739771 ) ) ;
#30118=CARTESIAN_POINT ( 'NONE',  ( -94.45264787283750252, -297.3609209418207229, -224.8931110739979147 ) ) ;
#30121=CARTESIAN_POINT ( 'NONE',  ( -112.3338901535364300, -280.3492042132492656, -280.0201395498779107 ) ) ;
#30123=CARTESIAN_POINT ( 'NONE',  ( -109.1929490945742174, -279.8237491719950185, -255.7507178831741612 ) ) ;
#30124=CARTESIAN_POINT ( 'NONE',  ( -98.62409087331593582, -280.9171217818589525, -225.4120688187577173 ) ) ;
#30125=CARTESIAN_POINT ( 'NONE',  ( -46.24351805935556570, -272.4170462749300441, -197.2074072826019631 ) ) ;
#30128=CARTESIAN_POINT ( 'NONE',  ( -89.47506570765176548, -279.4591624156437888, -219.1904344299709919 ) ) ;
#30129=CARTESIAN_POINT ( 'NONE',  ( 39.22047409388549966, -276.4365822727612567, -276.8720548231434009 ) ) ;
#30130=CARTESIAN_POINT ( 'NONE',  ( 37.15421243576869159, -277.6693848272579430, -279.4788039863135509 ) ) ;
#30131=CARTESIAN_POINT ( 'NONE',  ( -108.1175415534468129, -276.7583173844070643, -299.1601902256080052 ) ) ;
#30134=CARTESIAN_POINT ( 'NONE',  ( -27.56008033704150151, -284.9085126768122223, -345.1309870343359307 ) ) ;
#30135=CARTESIAN_POINT ( 'NONE',  ( -79.61569437200199673, -290.6619683924230912, -210.5871261692188909 ) ) ;
#30136=CARTESIAN_POINT ( 'NONE',  ( 38.19162196685588384, -286.7201203067720030, -255.9378714625147779 ) ) ;
#30137=CARTESIAN_POINT ( 'NONE',  ( -48.50331597433281416, -281.4360380136679396, -343.5279980811232576 ) ) ;
#30138=CARTESIAN_POINT ( 'NONE',  ( 18.03639702554986002, -280.8128498098408841, -318.8239003397196711 ) ) ;
#30139=AXIS2_PLACEMENT_3D ( 'NONE', #81494, #37478, #1504 ) ;
#30140=CARTESIAN_POINT ( 'NONE',  ( 21.63894991998256145, -282.1477639851155459, -226.6545790307598054 ) ) ;
#30141=CARTESIAN_POINT ( 'NONE',  ( -86.70047571675702613, -271.3662507222570639, -213.8234097619546219 ) ) ;
#30142=CARTESIAN_POINT ( 'NONE',  ( -67.58279608179554998, -281.8422218276042486, -340.3033550954222051 ) ) ;
#30143=CARTESIAN_POINT ( 'NONE',  ( 7.725231197364196056, -296.4369795947166608, -330.3108664946351496 ) ) ;
#30144=CARTESIAN_POINT ( 'NONE',  ( -109.3851267025530092, -279.0393106004819970, -282.8301124329083223 ) ) ;
#30145=CARTESIAN_POINT ( 'NONE',  ( -33.83886628530915175, -288.0962950638214579, -195.2761089353646469 ) ) ;
#30147=CARTESIAN_POINT ( 'NONE',  ( -71.54276086448386707, -293.5241592926616363, -202.9702239270277175 ) ) ;
#30148=CARTESIAN_POINT ( 'NONE',  ( 32.12099931849648016, -273.9223669930391338, -298.7822961012818723 ) ) ;
#30149=CARTESIAN_POINT ( 'NONE',  ( 23.15398890556640055, -287.3841174119747848, -317.7577206832503407 ) ) ;
#30150=CARTESIAN_POINT ( 'NONE',  ( 35.27396229666292271, -291.7792723841939733, -257.1223715479595171 ) ) ;
#30151=CARTESIAN_POINT ( 'NONE',  ( -93.11172295067521532, -276.5601329371263546, -318.2249669027065124 ) ) ;
#30152=CARTESIAN_POINT ( 'NONE',  ( -97.87648114938544097, -295.2818006853650559, -227.3912940564206053 ) ) ;
#30153=CARTESIAN_POINT ( 'NONE',  ( -110.7392158005492746, -291.9281324911635807, -265.7210610091478884 ) ) ;
#30156=CARTESIAN_POINT ( 'NONE',  ( -83.77875105064504169, -294.1561104215476803, -330.9777971006653274 ) ) ;
#30157=CARTESIAN_POINT ( 'NONE',  ( -6.702765334347680515, -288.0613556947406551, -203.2078647832507556 ) ) ;
#30158=CARTESIAN_POINT ( 'NONE',  ( -76.62593400905898022, -289.7743471410888105, -205.2564361816217513 ) ) ;
#30160=CARTESIAN_POINT ( 'NONE',  ( -61.43089932668555520, -290.7965654293739703, -339.8958963207621764 ) ) ;
#30162=CARTESIAN_POINT ( 'NONE',  ( -106.1810578772126803, -291.0257658261553502, -295.1349863008159105 ) ) ;
#30163=CARTESIAN_POINT ( 'NONE',  ( 82.70991478241074901, -294.7622393454342955, -192.9651424135201978 ) ) ;
#30164=CARTESIAN_POINT ( 'NONE',  ( 22.10675684709861244, -289.4088910859131829, -318.6921149016038726 ) ) ;
#30165=CARTESIAN_POINT ( 'NONE',  ( -42.29618563562885214, -278.0100698489151227, -195.1689649544283327 ) ) ;
#30166=CARTESIAN_POINT ( 'NONE',  ( -110.5309065621770799, -279.1875282015388393, -246.3364178433875793 ) ) ;
#30167=CARTESIAN_POINT ( 'NONE',  ( -53.75183047952486959, -279.5139571177062408, -195.0971774618754182 ) ) ;
#30168=CARTESIAN_POINT ( 'NONE',  ( -24.78250194733549350, -284.2120783827820674, -196.3674413647481458 ) ) ;
#30170=CARTESIAN_POINT ( 'NONE',  ( -41.09025825814673993, -278.1440525598329145, -196.2206176219276870 ) ) ;
#30171=CARTESIAN_POINT ( 'NONE',  ( -93.84520406591781239, -281.8672429109765858, -319.6800260566835163 ) ) ;
#30172=LINE ( 'NONE', #44826, #47208 ) ;
#30173=CARTESIAN_POINT ( 'NONE',  ( -92.55855033101936158, -277.7593677169328998, -217.6186982404646244 ) ) ;
#30174=CARTESIAN_POINT ( 'NONE',  ( -97.45945384162361336, -298.6617925869351211, -227.7399560822100000 ) ) ;
#30175=CARTESIAN_POINT ( 'NONE',  ( -113.5110258901397344, -283.5846025298166069, -261.4321582250794904 ) ) ;
#30176=CARTESIAN_POINT ( 'NONE',  ( -104.5320494842226111, -273.7446695103117236, -241.2834475317601459 ) ) ;
#30177=CARTESIAN_POINT ( 'NONE',  ( -69.89734441942776755, -275.0570847431282004, -201.2184090894064070 ) ) ;
#30178=CARTESIAN_POINT ( 'NONE',  ( 13.74308875761833626, -275.9788964967798393, -322.6084621437045143 ) ) ;
#30179=CARTESIAN_POINT ( 'NONE',  ( -25.87723045760135676, -296.9062861080032576, -344.4797160644679366 ) ) ;
#30180=CARTESIAN_POINT ( 'NONE',  ( -71.90456699023603448, -289.6631102814326937, -339.1681542419446487 ) ) ;
#30181=CARTESIAN_POINT ( 'NONE',  ( -28.37122901962571220, -278.2448237657351910, -195.2828666228588474 ) ) ;
#30182=CARTESIAN_POINT ( 'NONE',  ( -98.16091188482273822, -289.7548223246985231, -317.5842424643398658 ) ) ;
#30183=CARTESIAN_POINT ( 'NONE',  ( -109.4125984186034941, -289.4398581837099300, -283.3685800013030871 ) ) ;
#30184=CARTESIAN_POINT ( 'NONE',  ( 14.08579696907419176, -290.7735027733177731, -215.6984578696483936 ) ) ;
#30187=CARTESIAN_POINT ( 'NONE',  ( -84.72970518872624268, -289.2334503304113582, -326.0369406580814484 ) ) ;
#30189=CARTESIAN_POINT ( 'NONE',  ( -64.47527094818114790, -286.6477594083775671, -198.5375953359388745 ) ) ;
#30190=CARTESIAN_POINT ( 'NONE',  ( -82.13390479932378696, -293.9090924074131408, -214.2458315076590907 ) ) ;
#30191=CARTESIAN_POINT ( 'NONE',  ( -50.43920591083087146, -294.2740786875986601, -346.0540131091070748 ) ) ;
#30192=CARTESIAN_POINT ( 'NONE',  ( -47.17627517790656100, -284.4897857653093070, -346.2332433351776899 ) ) ;
#30193=CARTESIAN_POINT ( 'NONE',  ( -71.17633621112906894, -285.4256853905133084, -205.6755909641199196 ) ) ;
#30194=CARTESIAN_POINT ( 'NONE',  ( -0.3121701844103375589, -275.8707821412817225, -206.8636972637348777 ) ) ;
#30195=CARTESIAN_POINT ( 'NONE',  ( 22.63331556080247964, -292.1816536754992626, -314.8003382543167845 ) ) ;
#30196=CARTESIAN_POINT ( 'NONE',  ( -74.46101864683414817, -272.3419033558187721, -206.9833213208681002 ) ) ;
#30199=CARTESIAN_POINT ( 'NONE',  ( -1.980971705058676147, -294.2634876193852733, -338.7377454001368733 ) ) ;
#30200=CARTESIAN_POINT ( 'NONE',  ( 7.780754051210105438, -288.5934833683622855, -211.0906157817430540 ) ) ;
#30201=CARTESIAN_POINT ( 'NONE',  ( -113.9242464031971167, -297.5693897968903343, -275.3330899628325028 ) ) ;
#30202=CARTESIAN_POINT ( 'NONE',  ( 34.66634369526079951, -288.0338391656661088, -257.4767836045377294 ) ) ;
#30203=CARTESIAN_POINT ( 'NONE',  ( -112.7627509267349666, -277.7911728209131752, -255.9910392694391135 ) ) ;
#30204=CARTESIAN_POINT ( 'NONE',  ( -36.26754100742733300, -295.6904630566978653, -347.2647691543587030 ) ) ;
#30205=CARTESIAN_POINT ( 'NONE',  ( 22.30021413210127434, -286.3267052447318406, -317.1061646440770119 ) ) ;
#30207=CARTESIAN_POINT ( 'NONE',  ( 38.04033725231291641, -293.6894974325553562, -254.6986855815668207 ) ) ;
#30211=CARTESIAN_POINT ( 'NONE',  ( 13.76800080992791209, -288.2730208979230611, -213.6289157487942134 ) ) ;
#30212=CARTESIAN_POINT ( 'NONE',  ( -37.30987171927208834, -283.5523547857346784, -190.3611179825600175 ) ) ;
#30214=CARTESIAN_POINT ( 'NONE',  ( -72.45286105436480284, -278.9484061160697479, -201.9321668036308779 ) ) ;
#30215=CARTESIAN_POINT ( 'NONE',  ( 36.84695773332270363, -283.4212380202399117, -260.1752286230858999 ) ) ;
#30216=CARTESIAN_POINT ( 'NONE',  ( -109.5359067363892649, -271.2847351524787882, -295.9514105794971215 ) ) ;
#30217=CARTESIAN_POINT ( 'NONE',  ( -111.6504275734346692, -282.9018657936875343, -288.2159785687240401 ) ) ;
#30218=CARTESIAN_POINT ( 'NONE',  ( 35.69229606948139377, -285.8191291156263105, -284.8265420699412971 ) ) ;
#30219=CARTESIAN_POINT ( 'NONE',  ( 27.43400751626292333, -276.8900371757659400, -230.9618491059271435 ) ) ;
#30220=CARTESIAN_POINT ( 'NONE',  ( -109.3375671564939324, -297.2083773113723737, -257.9279537597230387 ) ) ;
#30222=CARTESIAN_POINT ( 'NONE',  ( -31.58029224352640441, -293.6628608937987792, -343.6785451164006417 ) ) ;
#30223=CARTESIAN_POINT ( 'NONE',  ( -111.3401656600164813, -278.9410550708571463, -291.2785720742067497 ) ) ;
#30224=CARTESIAN_POINT ( 'NONE',  ( 20.83691996384193601, -276.1717946529852270, -314.4547475020229967 ) ) ;
#30225=CARTESIAN_POINT ( 'NONE',  ( -83.40544964237400904, -274.5173070286849679, -208.9788751809859377 ) ) ;
#30226=CARTESIAN_POINT ( 'NONE',  ( -99.40772545839395491, -276.8721704488895625, -315.4312170439667966 ) ) ;
#30227=CARTESIAN_POINT ( 'NONE',  ( 5.216678999390555127, -58.13084686240627263, -354.5881712518564655 ) ) ;
#30228=CARTESIAN_POINT ( 'NONE',  ( 36.53642750459122368, -273.3851100515191206, -257.3639452198239610 ) ) ;
#30230=CARTESIAN_POINT ( 'NONE',  ( -99.51837872833381482, -297.3835110046858858, -314.8649253165854702 ) ) ;
#30233=CARTESIAN_POINT ( 'NONE',  ( -95.20949855451260646, -286.2634741874908286, -225.3346861841081648 ) ) ;
#30234=CARTESIAN_POINT ( 'NONE',  ( -67.45883343092104667, -285.2019483794857138, -340.1245202582179559 ) ) ;
#30235=CARTESIAN_POINT ( 'NONE',  ( 22.07927720021442042, -286.3054152180918663, -227.6959539942548076 ) ) ;
#30236=CARTESIAN_POINT ( 'NONE',  ( -111.1925598651727825, -276.9486279954259658, -270.6207518743560740 ) ) ;
#30237=CARTESIAN_POINT ( 'NONE',  ( -111.2262055364654003, -286.5126709601237849, -262.6448169906840917 ) ) ;
#30238=CARTESIAN_POINT ( 'NONE',  ( -32.90208420742211359, -278.5889754397038018, -196.8016348164179021 ) ) ;
#30239=CARTESIAN_POINT ( 'NONE',  ( -48.64197946262460448, -278.2789591126079358, -342.8456560869590817 ) ) ;
#30241=CARTESIAN_POINT ( 'NONE',  ( 51.81736995740534013, -299.8487276833988631, -197.2490443897613375 ) ) ;
#30242=CARTESIAN_POINT ( 'NONE',  ( 37.17215754845398834, -282.1197936335277063, -251.6036172092029233 ) ) ;
#30243=CARTESIAN_POINT ( 'NONE',  ( 25.06105409695339858, -282.6419452536333097, -315.3881858004331207 ) ) ;
#30247=CARTESIAN_POINT ( 'NONE',  ( 17.44171303467886602, -288.6844726397104637, -217.9492308230940978 ) ) ;
#30248=CARTESIAN_POINT ( 'NONE',  ( -112.3875668390121092, -289.0488516162957353, -285.3076532172833026 ) ) ;
#30249=CARTESIAN_POINT ( 'NONE',  ( -52.65894066684864327, -297.0481588155813597, -198.7690334284515075 ) ) ;
#30250=CARTESIAN_POINT ( 'NONE',  ( 4.093605395896895871, -291.9429946030872998, -205.5181527295502804 ) ) ;
#30251=CARTESIAN_POINT ( 'NONE',  ( -0.6630064052688882104, -287.0356768691353295, -334.3368343582113198 ) ) ;
#30252=CARTESIAN_POINT ( 'NONE',  ( -45.44521468341863368, -287.7315611833651019, -343.5028158608826629 ) ) ;
#30253=CARTESIAN_POINT ( 'NONE',  ( -42.71844824893391745, -287.1879180690430076, -197.1485528861257990 ) ) ;
#30254=CARTESIAN_POINT ( 'NONE',  ( -110.1383538744669579, -276.7843817836933340, -252.2627859587048249 ) ) ;
#30255=CARTESIAN_POINT ( 'NONE',  ( 37.10853860683869954, -289.6740782642317527, -279.8443553187082102 ) ) ;
#30256=CARTESIAN_POINT ( 'NONE',  ( -0.2090916398011355148, -286.5597075687548454, -335.7743283815552786 ) ) ;
#30257=CARTESIAN_POINT ( 'NONE',  ( -99.81628277745228672, -286.0194206094087122, -232.0501431294695465 ) ) ;
#30258=CARTESIAN_POINT ( 'NONE',  ( -111.3709646190213221, -292.7192025155866304, -257.3343598552531262 ) ) ;
#30261=CARTESIAN_POINT ( 'NONE',  ( -36.58377548792454803, -299.9817177801803609, -194.8008643405604232 ) ) ;
#30262=CARTESIAN_POINT ( 'NONE',  ( -38.34581969193056494, -279.2364166948810862, -197.1941039448001334 ) ) ;
#30263=CARTESIAN_POINT ( 'NONE',  ( 15.31110376582103783, -280.3087349713057392, -323.8447278044608311 ) ) ;
#30264=CARTESIAN_POINT ( 'NONE',  ( 38.69363438383049214, -292.6059706856769935, -258.9228752454965274 ) ) ;
#30265=CARTESIAN_POINT ( 'NONE',  ( -33.74297281102408874, -296.4978057387346553, -196.5621124728592122 ) ) ;
#30266=CARTESIAN_POINT ( 'NONE',  ( -24.09694663086387223, -274.9616789924215254, -343.6658215369304230 ) ) ;
#30267=CARTESIAN_POINT ( 'NONE',  ( -90.41350849308709314, -298.5967181987629715, -219.4490461642845673 ) ) ;
#30269=CARTESIAN_POINT ( 'NONE',  ( -60.67379830528999918, -272.3301244463054900, -197.5445312275051037 ) ) ;
#30270=CARTESIAN_POINT ( 'NONE',  ( -110.2495387628530779, -294.5193444744269300, -291.8178300790127651 ) ) ;
#30271=CARTESIAN_POINT ( 'NONE',  ( 33.32101971620121361, -295.2475691219497094, -290.9528583762774474 ) ) ;
#30273=CARTESIAN_POINT ( 'NONE',  ( -7.913995945544356481, -295.4592964853624153, -337.3569028352923738 ) ) ;
#30276=CARTESIAN_POINT ( 'NONE',  ( -63.94246463210787113, -283.7270864277783744, -199.8433109332171682 ) ) ;
#30277=CARTESIAN_POINT ( 'NONE',  ( -93.61357235408382849, -297.2115686369666037, -223.8392375785866477 ) ) ;
#30278=CARTESIAN_POINT ( 'NONE',  ( -83.88320362439178268, -283.6712409306389304, -331.7704834050782665 ) ) ;
#30279=CARTESIAN_POINT ( 'NONE',  ( 38.09326361532798444, -283.5382781509355823, -275.5374234817456909 ) ) ;
#30281=CARTESIAN_POINT ( 'NONE',  ( -76.09240538327740921, -285.2162828544068134, -203.7856241204926562 ) ) ;
#30282=CARTESIAN_POINT ( 'NONE',  ( 14.18346396892100891, -290.7778141388332642, -216.0915511023330851 ) ) ;
#30284=CARTESIAN_POINT ( 'NONE',  ( -112.9668995883443046, -277.7253469392597935, -284.3669904164597142 ) ) ;
#30286=CARTESIAN_POINT ( 'NONE',  ( 31.98288692825982693, -278.6237833571633473, -237.0123917617630980 ) ) ;
#30288=CARTESIAN_POINT ( 'NONE',  ( 11.40919638131766334, -285.5406086466460351, -215.4249723980004774 ) ) ;
#30289=CARTESIAN_POINT ( 'NONE',  ( -103.5385905743978299, -288.9652926162976883, -309.1891042702944219 ) ) ;
#30291=CARTESIAN_POINT ( 'NONE',  ( -113.4586770934678981, -280.0690816424614695, -263.0882024961543380 ) ) ;
#30292=CARTESIAN_POINT ( 'NONE',  ( 20.99690167611707992, -292.2267308071288880, -318.0784761412790544 ) ) ;
#30293=CARTESIAN_POINT ( 'NONE',  ( 31.37305291535080798, -281.5495801154356172, -295.2162674044034247 ) ) ;
#30294=CARTESIAN_POINT ( 'NONE',  ( -27.74572995558257205, -295.1003075988508044, -346.8141314721231083 ) ) ;
#30295=CARTESIAN_POINT ( 'NONE',  ( -0.3984978190463963066, -284.6190928866167269, -204.4334220869432386 ) ) ;
#30296=CARTESIAN_POINT ( 'NONE',  ( -81.09334692990802296, -281.4579206211412838, -209.4448307667076392 ) ) ;
#30298=CARTESIAN_POINT ( 'NONE',  ( -84.63917256563671287, -294.7810418449220151, -326.3415515476017958 ) ) ;
#30299=CARTESIAN_POINT ( 'NONE',  ( -21.02729779183863457, -296.2562167332568492, -195.3666715009129291 ) ) ;
#30302=CARTESIAN_POINT ( 'NONE',  ( 20.08572133293977302, -282.8704095424396883, -222.6554623309425835 ) ) ;
#30303=CARTESIAN_POINT ( 'NONE',  ( -82.40268784573207483, -295.1938603393234075, -327.9364573860551673 ) ) ;
#30304=CARTESIAN_POINT ( 'NONE',  ( -4.771743288812454686, -277.9809262143061233, -202.8022627189028810 ) ) ;
#30305=CARTESIAN_POINT ( 'NONE',  ( 15.92247725145063164, -273.9813353613054687, -214.9798374967508039 ) ) ;
#30306=CARTESIAN_POINT ( 'NONE',  ( -94.95187638088701476, -289.7535825356361556, -315.2150918889023501 ) ) ;
#30307=CARTESIAN_POINT ( 'NONE',  ( -35.66626166038895462, -281.5936407158752104, -196.6743094552464584 ) ) ;
#30308=CARTESIAN_POINT ( 'NONE',  ( -36.74990220974716948, -275.6598393021289439, -196.5509373181357944 ) ) ;
#30309=CARTESIAN_POINT ( 'NONE',  ( -63.61684283494066250, -284.9891515630255867, -341.8877374373977887 ) ) ;
#30310=CARTESIAN_POINT ( 'NONE',  ( -46.49082093992373643, -278.7285195091731680, -197.4851269918347327 ) ) ;
#30311=CARTESIAN_POINT ( 'NONE',  ( -2.927673812715636537, -278.5974601240934021, -336.9995111557383893 ) ) ;
#30313=CARTESIAN_POINT ( 'NONE',  ( -92.16757407084827491, -273.1281190401284107, -216.2951994116943979 ) ) ;
#30314=CARTESIAN_POINT ( 'NONE',  ( -103.7041911062083415, -292.9227972320578033, -236.5225566655315959 ) ) ;
#30315=DIRECTION ( 'NONE',  ( -1.000000000000000000, -0.000000000000000000, -0.000000000000000000 ) ) ;
#30317=CARTESIAN_POINT ( 'NONE',  ( 20.41049706642102635, -292.3636173436287322, -319.4018072343007475 ) ) ;
#30318=CARTESIAN_POINT ( 'NONE',  ( -29.97743445099836990, -273.6555251594185734, -197.6716687297717669 ) ) ;
#30320=CARTESIAN_POINT ( 'NONE',  ( -3.645126016569865346, -294.0088408306101542, -201.8832293386361982 ) ) ;
#30321=CARTESIAN_POINT ( 'NONE',  ( 31.95455697924148097, -277.6233781216988064, -236.9535640164627637 ) ) ;
#30322=CARTESIAN_POINT ( 'NONE',  ( -39.21743087396442462, -293.2342056103323671, -193.7681896800372954 ) ) ;
#30323=CARTESIAN_POINT ( 'NONE',  ( -10.10587582712289390, -288.4086670888771096, -200.6461907207715001 ) ) ;
#30324=CARTESIAN_POINT ( 'NONE',  ( 36.17933434339929732, -273.3724385954732270, -256.4081283615719826 ) ) ;
#30325=CARTESIAN_POINT ( 'NONE',  ( 32.62343200360369622, -277.8062046725396499, -295.9314017754524002 ) ) ;
#30326=CARTESIAN_POINT ( 'NONE',  ( -31.51353581329227538, -293.0579784533805423, -344.6237197267218448 ) ) ;
#30327=CARTESIAN_POINT ( 'NONE',  ( -106.3048038756326434, -280.8215654241241737, -238.8596333688762741 ) ) ;
#30329=CARTESIAN_POINT ( 'NONE',  ( -48.33605347603156588, -282.8626682788591324, -342.5498406556216082 ) ) ;
#30330=CARTESIAN_POINT ( 'NONE',  ( -42.42335529951948558, -281.0691395003895536, -193.8387729409524525 ) ) ;
#30331=CARTESIAN_POINT ( 'NONE',  ( -63.78939666134351683, -282.1843998303464218, -342.2535937109928454 ) ) ;
#30332=CARTESIAN_POINT ( 'NONE',  ( -22.97115700840193497, -277.8140107069497731, -345.8227490489386469 ) ) ;
#30333=CARTESIAN_POINT ( 'NONE',  ( 35.83413559433095230, -277.3466603205235970, -292.0406781009871793 ) ) ;
#30334=CIRCLE ( 'NONE', #83245, 6.654241149514406040 ) ;
#30335=CARTESIAN_POINT ( 'NONE',  ( -21.39648532958013050, -288.7662352645559167, -200.3538533559491555 ) ) ;
#30337=CARTESIAN_POINT ( 'NONE',  ( -111.0149742419033601, -298.7335213469509085, -256.2480504441812172 ) ) ;
#30339=CARTESIAN_POINT ( 'NONE',  ( -55.10048773536283306, -292.8980161745895998, -199.2355140457789844 ) ) ;
#30340=CARTESIAN_POINT ( 'NONE',  ( -81.81920467862833846, -275.6815405491170736, -330.3077474851269812 ) ) ;
#30341=CARTESIAN_POINT ( 'NONE',  ( -31.87697628902859392, -290.7443628320071980, -346.2028942339384230 ) ) ;
#30342=CARTESIAN_POINT ( 'NONE',  ( -70.25919855877152997, -290.9549519717219823, -205.0899071343594073 ) ) ;
#30343=CARTESIAN_POINT ( 'NONE',  ( 39.54250020041620672, -287.1106828574784231, -274.4259407631919885 ) ) ;
#30345=CARTESIAN_POINT ( 'NONE',  ( -107.7551894163143942, -282.6622909905218535, -292.4604605435873736 ) ) ;
#30346=CARTESIAN_POINT ( 'NONE',  ( -102.7199382873946831, -291.9397190867373411, -305.6346748019720962 ) ) ;
#30347=CARTESIAN_POINT ( 'NONE',  ( -105.8657154033121230, -282.6711072155442821, -297.6140826549684562 ) ) ;
#30348=CARTESIAN_POINT ( 'NONE',  ( -37.02288509367984659, -281.3714029382598483, -196.8686568953267226 ) ) ;
#30349=ORIENTED_EDGE ( 'NONE', *, *, #76250, .F. ) ;
#30350=CARTESIAN_POINT ( 'NONE',  ( -41.73507411098987063, -290.0474468415446267, -347.0131833871716367 ) ) ;
#30351=CARTESIAN_POINT ( 'NONE',  ( -104.5010969102864209, -279.4306298667779060, -241.5930129818785588 ) ) ;
#30352=CARTESIAN_POINT ( 'NONE',  ( -56.07674356019526130, -290.6111059782531925, -196.0298997386839517 ) ) ;
#30353=CARTESIAN_POINT ( 'NONE',  ( -4.851538190235796577, -287.2720583852579921, -200.7296007040601751 ) ) ;
#30354=CARTESIAN_POINT ( 'NONE',  ( 31.36402371041186043, -287.5985563649752521, -235.7338106242785614 ) ) ;
#30355=CARTESIAN_POINT ( 'NONE',  ( -73.55747563525513044, -285.7238955599361816, -206.9635197812090155 ) ) ;
#30358=CARTESIAN_POINT ( 'NONE',  ( -2.642990226368007178, -294.3663695353113212, -202.9944820103840470 ) ) ;
#30359=CARTESIAN_POINT ( 'NONE',  ( -19.41916274868404457, -293.5112345375185896, -344.7936092943125459 ) ) ;
#30360=CARTESIAN_POINT ( 'NONE',  ( 0.9843800942212024285, -275.5861474456087876, -332.8267897707962675 ) ) ;
#30361=CARTESIAN_POINT ( 'NONE',  ( -29.06492020340282778, -297.5018191483918599, -193.4639370183433016 ) ) ;
#30362=CARTESIAN_POINT ( 'NONE',  ( 35.40143388415661718, -291.8768489228952490, -258.4861426334520047 ) ) ;
#30363=CARTESIAN_POINT ( 'NONE',  ( -82.54553853620640780, -295.6652607265676806, -211.6908282022216952 ) ) ;
#30364=CARTESIAN_POINT ( 'NONE',  ( -103.9229279011404117, -292.1719071713685594, -239.4730845091687002 ) ) ;
#30365=CARTESIAN_POINT ( 'NONE',  ( 35.21170535592063544, -294.4939126146782087, -259.8620977229191453 ) ) ;
#30367=CARTESIAN_POINT ( 'NONE',  ( 29.26571745237979982, -292.0124013390278037, -305.1961627919250759 ) ) ;
#30368=CARTESIAN_POINT ( 'NONE',  ( -111.4943479972778277, -298.7009193367680382, -258.7873342821916935 ) ) ;
#30369=CARTESIAN_POINT ( 'NONE',  ( -109.5107109708226574, -291.6609480034854300, -257.6197056666317735 ) ) ;
#30370=CARTESIAN_POINT ( 'NONE',  ( -39.68546534238544865, -295.4156426965833475, -343.3570724978961266 ) ) ;
#30371=CARTESIAN_POINT ( 'NONE',  ( -96.61908903814438077, -279.8964643142735440, -316.8863581359638033 ) ) ;
#30372=CARTESIAN_POINT ( 'NONE',  ( -105.7272149595642077, -277.6824318132854614, -235.9398308455830318 ) ) ;
#30374=CARTESIAN_POINT ( 'NONE',  ( -55.30175408553317595, -273.1755397483860861, -195.5898049800782417 ) ) ;
#30375=CARTESIAN_POINT ( 'NONE',  ( 19.07149728193752836, -278.9535283398895444, -221.7733912578554225 ) ) ;
#30376=CARTESIAN_POINT ( 'NONE',  ( -113.2836809559127715, -276.8651125563465598, -277.2383869981181306 ) ) ;
#30377=CARTESIAN_POINT ( 'NONE',  ( -109.9532474719436692, -276.8018089361800094, -250.8797735318345019 ) ) ;
#30378=CARTESIAN_POINT ( 'NONE',  ( -36.45929366230426893, -296.7482493882942549, -196.8681658811741215 ) ) ;
#30381=CARTESIAN_POINT ( 'NONE',  ( -78.67078869881135006, -289.5190210015192065, -207.2883347966385941 ) ) ;
#30382=CARTESIAN_POINT ( 'NONE',  ( -100.6805982995358590, -289.9739069087532357, -314.1467774891395379 ) ) ;
#30383=CARTESIAN_POINT ( 'NONE',  ( -34.20579486126489144, -276.0916655262454356, -195.2598894506807596 ) ) ;
#30384=CARTESIAN_POINT ( 'NONE',  ( -86.60518985941068593, -271.3678742410480709, -213.7400918087003276 ) ) ;
#30386=CARTESIAN_POINT ( 'NONE',  ( -47.24569550462377521, -282.3721204272555383, -346.5586881259623055 ) ) ;
#30389=CARTESIAN_POINT ( 'NONE',  ( -68.76226250186361710, -281.4649774995575626, -338.4759357310989003 ) ) ;
#30391=CARTESIAN_POINT ( 'NONE',  ( 34.03750243871256487, -292.1221611069201458, -253.2152750703466211 ) ) ;
#30392=CARTESIAN_POINT ( 'NONE',  ( -103.3256569276116608, -283.1464602072390448, -236.3466663095536830 ) ) ;
#30395=CARTESIAN_POINT ( 'NONE',  ( 35.04037714199228759, -291.8051198903942236, -290.0525820121833362 ) ) ;
#30396=CARTESIAN_POINT ( 'NONE',  ( -102.5544251687881285, -279.6867336996780864, -304.9116737804314425 ) ) ;
#30397=CARTESIAN_POINT ( 'NONE',  ( 6.709278043402101765, -283.6731277203155628, -333.0959205434032242 ) ) ;
#30398=CARTESIAN_POINT ( 'NONE',  ( -89.15725053474784545, -271.4104081430577935, -215.2945728974029862 ) ) ;
#30399=CARTESIAN_POINT ( 'NONE',  ( -30.53128379256239811, -286.1405258354367902, -197.6286971215307915 ) ) ;
#30400=CARTESIAN_POINT ( 'NONE',  ( 33.81656149352531315, -277.2231388504179108, -289.1194953492233140 ) ) ;
#30401=CARTESIAN_POINT ( 'NONE',  ( -6.198624515589422401, -277.4349988267793492, -336.5769615598744053 ) ) ;
#30402=CARTESIAN_POINT ( 'NONE',  ( -84.28153266069087124, -287.4065314959399302, -211.8662227571742847 ) ) ;
#30405=CARTESIAN_POINT ( 'NONE',  ( -104.6039383322747511, -295.8983334081426619, -307.9506680985916773 ) ) ;
#30407=CARTESIAN_POINT ( 'NONE',  ( 34.97595073988657077, -289.2927182412562388, -251.8162419054780798 ) ) ;
#30408=DIRECTION ( 'NONE',  ( 1.000000000000000000, 0.000000000000000000, 0.000000000000000000 ) ) ;
#30409=CARTESIAN_POINT ( 'NONE',  ( 13.84574458161073807, -290.1952119285918457, -206.2264541496106460 ) ) ;
#30410=CARTESIAN_POINT ( 'NONE',  ( -112.4121188193232967, -277.6701916319069596, -254.6158561427491236 ) ) ;
#30411=CARTESIAN_POINT ( 'NONE',  ( -44.79826888974096732, -290.3592740396309750, -194.4744527159748486 ) ) ;
#30412=CARTESIAN_POINT ( 'NONE',  ( -107.6415148815863745, -285.7820378585417416, -292.4664069034336649 ) ) ;
#30413=CARTESIAN_POINT ( 'NONE',  ( -62.67659069883896450, -281.4781417358979638, -200.7648144946293769 ) ) ;
#30414=CARTESIAN_POINT ( 'NONE',  ( 38.76222251870924396, -289.0636382209721660, -277.2021156870180789 ) ) ;
#30415=CARTESIAN_POINT ( 'NONE',  ( -6.405871439189798622, -284.6460189565929682, -338.6977914707035779 ) ) ;
#30416=CARTESIAN_POINT ( 'NONE',  ( 5.873036110653372610, -276.6503655297937598, -334.0909114570975476 ) ) ;
#30417=CARTESIAN_POINT ( 'NONE',  ( -112.0163699347023254, -270.6241775036895660, -264.7512697947053653 ) ) ;
#30418=CARTESIAN_POINT ( 'NONE',  ( -31.07164192017774695, -279.9624873919271408, -193.5641351461285069 ) ) ;
#30419=CARTESIAN_POINT ( 'NONE',  ( -110.4647240449685768, -298.6535278541505818, -256.3526129439659371 ) ) ;
#30422=CARTESIAN_POINT ( 'NONE',  ( -101.8468313567045271, -271.3244763921799745, -230.1981741443804026 ) ) ;
#30424=CARTESIAN_POINT ( 'NONE',  ( -24.85971845886106379, -279.7233467573310008, -198.3736984212217749 ) ) ;
#30425=CARTESIAN_POINT ( 'NONE',  ( -1.639118197081272932, -277.7946757131378490, -338.1352602714663931 ) ) ;
#30426=CARTESIAN_POINT ( 'NONE',  ( -88.17472866643004181, -282.8018551907403548, -327.9544767035242785 ) ) ;
#30427=CARTESIAN_POINT ( 'NONE',  ( -80.98723948211757317, -291.4137133836126168, -330.1997979591640728 ) ) ;
#30428=CARTESIAN_POINT ( 'NONE',  ( 75.09555894462938852, -300.9558628955291510, -194.0259358155473137 ) ) ;
#30429=CARTESIAN_POINT ( 'NONE',  ( -84.98152943331974996, -298.6163183540284649, -210.3739911866694854 ) ) ;
#30430=CARTESIAN_POINT ( 'NONE',  ( -9.057584995526280380, -294.4228991617147813, -201.0236906152386211 ) ) ;
#30431=CARTESIAN_POINT ( 'NONE',  ( 29.78460333268899163, -279.9906237201117278, -303.5556337500761970 ) ) ;
#30432=CARTESIAN_POINT ( 'NONE',  ( -45.77886591144952888, -285.0799528569187373, -344.3734333045267704 ) ) ;
#30433=CARTESIAN_POINT ( 'NONE',  ( 6.155220129386226091, -272.6653827330829927, -209.6353294603123345 ) ) ;
#30434=CARTESIAN_POINT ( 'NONE',  ( -92.83481871751310166, -285.4318179921757519, -322.6004883283499680 ) ) ;
#30435=CARTESIAN_POINT ( 'NONE',  ( -99.10958497953167523, -288.9286563528490888, -309.8447155189901991 ) ) ;
#30436=CARTESIAN_POINT ( 'NONE',  ( -82.85074041547900947, -220.2000674996521354, -352.4970221947974665 ) ) ;
#30438=CARTESIAN_POINT ( 'NONE',  ( -26.24817011758402785, -287.4883069314020076, -345.9623076794937333 ) ) ;
#30439=CARTESIAN_POINT ( 'NONE',  ( 33.10117376977922277, -287.4751140013740951, -289.7812115690613268 ) ) ;
#30441=CARTESIAN_POINT ( 'NONE',  ( -89.68535264957019137, -286.4144764689514773, -214.2385915595882011 ) ) ;
#30442=CARTESIAN_POINT ( 'NONE',  ( 32.91936102392261176, -276.1488043543715207, -290.2933326828679128 ) ) ;
#30443=CARTESIAN_POINT ( 'NONE',  ( 38.92812623901128433, -292.5793810875981080, -278.8742696593846517 ) ) ;
#30444=CARTESIAN_POINT ( 'NONE',  ( -13.44572669270460352, -283.4012094180182544, -343.4521245425622169 ) ) ;
#30445=CARTESIAN_POINT ( 'NONE',  ( 23.18541798193011161, -282.4465372654044586, -223.8728473738814273 ) ) ;
#30446=CARTESIAN_POINT ( 'NONE',  ( -38.72790996317126400, -283.4023727350203785, -347.3274918995299458 ) ) ;
#30447=CARTESIAN_POINT ( 'NONE',  ( 17.97777056028917642, -281.2065993437755083, -222.6780642741602492 ) ) ;
#30448=CARTESIAN_POINT ( 'NONE',  ( 31.95455697924147032, -273.4809262143061233, -303.7686719486574702 ) ) ;
#30449=CARTESIAN_POINT ( 'NONE',  ( 203.9605228849236482, 295.7236489450776276, -54.00000000003888800 ) ) ;
#30451=CARTESIAN_POINT ( 'NONE',  ( -111.7234250678460654, -280.4408017313708115, -279.0267913573229634 ) ) ;
#30452=CARTESIAN_POINT ( 'NONE',  ( -100.4790452129269056, -247.5007079388412308, -333.8973734642195836 ) ) ;
#30453=CARTESIAN_POINT ( 'NONE',  ( -110.2015576158204340, -295.8145898646614569, -276.9005189072779558 ) ) ;
#30454=CARTESIAN_POINT ( 'NONE',  ( 34.39185194042086380, -293.4125140408897323, -298.1788175771407055 ) ) ;
#30455=CARTESIAN_POINT ( 'NONE',  ( 45.91229879770529010, 10.79500447405072805, -328.5722265923597547 ) ) ;
#30456=CARTESIAN_POINT ( 'NONE',  ( 30.15906987437215747, -297.4563395728868613, -193.9663099215189277 ) ) ;
#30457=CARTESIAN_POINT ( 'NONE',  ( -109.9698033400114667, -288.7810882537460770, -283.4606996652667590 ) ) ;
#30458=CARTESIAN_POINT ( 'NONE',  ( -17.87414766398960353, -296.6588708410381514, -341.9982583410604775 ) ) ;
#30459=CARTESIAN_POINT ( 'NONE',  ( -35.94074817589108051, -287.3852644276557271, -196.8813193094359519 ) ) ;
#30461=CARTESIAN_POINT ( 'NONE',  ( -81.72585949647205439, -296.5811827581291595, -333.0588267331919496 ) ) ;
#30462=CARTESIAN_POINT ( 'NONE',  ( -83.69174465666141316, -285.8886752022341398, -213.8182881602106420 ) ) ;
#30463=CARTESIAN_POINT ( 'NONE',  ( -101.2101093160071628, -295.9065951526369531, -228.0426177672065933 ) ) ;
#30464=CARTESIAN_POINT ( 'NONE',  ( 30.75107741266623407, -293.8933821237206416, -234.6441807233576071 ) ) ;
#30465=CARTESIAN_POINT ( 'NONE',  ( 38.75660446740547371, -294.1864219334160566, -281.7002070524073361 ) ) ;
#30466=CARTESIAN_POINT ( 'NONE',  ( -38.89970730370525587, -292.1987465311190704, -197.3777457792164398 ) ) ;
#30469=CARTESIAN_POINT ( 'NONE',  ( -82.73489902193460921, -275.3576544430699187, -209.8905535330964369 ) ) ;
#30470=CARTESIAN_POINT ( 'NONE',  ( 34.35553623104942744, -274.0040781353523585, -243.3886316995457832 ) ) ;
#30471=ORIENTED_EDGE ( 'NONE', *, *, #57376, .T. ) ;
#30472=CARTESIAN_POINT ( 'NONE',  ( -56.91443260001816640, -276.8055402548901043, -344.8233523562348637 ) ) ;
#30473=CARTESIAN_POINT ( 'NONE',  ( -76.97689540850997503, -271.9112837363510380, -208.1076706127692262 ) ) ;
#30474=CARTESIAN_POINT ( 'NONE',  ( -100.5313930023285423, -280.9419870073729157, -231.3024050871305803 ) ) ;
#30475=CARTESIAN_POINT ( 'NONE',  ( 1.497822823686025151, -274.6671316817748334, -333.6856919576097198 ) ) ;
#30476=CARTESIAN_POINT ( 'NONE',  ( -32.68507366591525454, -275.1918596435633049, -197.1874703555207589 ) ) ;
#30477=CARTESIAN_POINT ( 'NONE',  ( -27.26964137307360403, -275.1244160056850774, -197.7706730866786415 ) ) ;
#30478=CARTESIAN_POINT ( 'NONE',  ( -68.44999301935921210, -275.4091918870223594, -201.0198003886684432 ) ) ;
#30480=CARTESIAN_POINT ( 'NONE',  ( -4.519241728081113685, -272.5025538490259009, -202.5155593285977602 ) ) ;
#30481=CARTESIAN_POINT ( 'NONE',  ( -31.58606522462891064, -295.6291308313591912, -343.2862990823888936 ) ) ;
#30482=CARTESIAN_POINT ( 'NONE',  ( 23.40924315264309996, -292.7012009180888299, -311.9796788935318546 ) ) ;
#30484=CARTESIAN_POINT ( 'NONE',  ( -7.902378773659134659, -277.1689944546349125, -341.4588164389803069 ) ) ;
#30485=CARTESIAN_POINT ( 'NONE',  ( 11.54494825625091003, -274.9194325188312291, -216.0796290706797720 ) ) ;
#30487=CARTESIAN_POINT ( 'NONE',  ( -73.36590380457026583, -284.2697656324123727, -202.8075956466740593 ) ) ;
#30488=CARTESIAN_POINT ( 'NONE',  ( -101.5363140113149427, -298.0292207621320131, -309.4645701748207784 ) ) ;
#30490=CARTESIAN_POINT ( 'NONE',  ( -35.92010057779749843, -285.2676005305355034, -197.2134537533384844 ) ) ;
#30491=CARTESIAN_POINT ( 'NONE',  ( -105.3578026010893609, -282.1321585602598248, -302.3585901925954431 ) ) ;
#30493=CARTESIAN_POINT ( 'NONE',  ( -109.8759070710191708, -276.9843959021232536, -255.5747007600660083 ) ) ;
#30494=CARTESIAN_POINT ( 'NONE',  ( -89.51628850626474332, -276.3795230077192286, -322.3294240728554314 ) ) ;
#30495=CARTESIAN_POINT ( 'NONE',  ( -70.86702211693705067, -281.6100788549769049, -203.2572118609458300 ) ) ;
#30496=CARTESIAN_POINT ( 'NONE',  ( -24.54219316581306387, -275.4240896212223220, -198.0368277259416914 ) ) ;
#30498=CARTESIAN_POINT ( 'NONE',  ( 5.405478655831243096, -274.8838416653731542, -333.4413773346328185 ) ) ;
#30499=CARTESIAN_POINT ( 'NONE',  ( -42.33433592278263546, -281.9894799696330665, -195.3604378836142814 ) ) ;
#30501=CARTESIAN_POINT ( 'NONE',  ( 25.91854806279937051, -288.9190693780342940, -229.0397530928516687 ) ) ;
#30502=CARTESIAN_POINT ( 'NONE',  ( -85.62563434231992687, -289.3844032141742559, -212.9036990776084508 ) ) ;
#30503=CARTESIAN_POINT ( 'NONE',  ( 82.12659874290375228, -301.3026828166021005, -196.3296339295530970 ) ) ;
#30504=CARTESIAN_POINT ( 'NONE',  ( -63.20509443755166501, -296.5026560326310801, -201.6180862338164559 ) ) ;
#30505=CARTESIAN_POINT ( 'NONE',  ( -67.03677985120376093, -289.7982920927141208, -202.3238655200340190 ) ) ;
#30506=CARTESIAN_POINT ( 'NONE',  ( -69.18520112214993389, -196.4157418647702968, -356.4528236438462159 ) ) ;
#30507=CARTESIAN_POINT ( 'NONE',  ( -33.66483702006775758, -296.0980222675469236, -195.3623628324206720 ) ) ;
#30508=CARTESIAN_POINT ( 'NONE',  ( 20.03863762098110612, -286.7189686795621242, -320.6819355527725293 ) ) ;
#30509=CARTESIAN_POINT ( 'NONE',  ( -82.65341198582420645, -283.6826963595871121, -209.2969704488729690 ) ) ;
#30510=CARTESIAN_POINT ( 'NONE',  ( -93.43983699933268383, -291.2150775458806038, -223.6297309859413076 ) ) ;
#30511=CARTESIAN_POINT ( 'NONE',  ( -1.696433660081715589, -281.9596978592288679, -205.9810752961918467 ) ) ;
#30512=CARTESIAN_POINT ( 'NONE',  ( 24.27194010876372232, -282.9006366957029854, -309.9050119520894100 ) ) ;
#30513=CARTESIAN_POINT ( 'NONE',  ( -23.58687808666093133, -290.8572269395274361, -344.5032935005667127 ) ) ;
#30514=CARTESIAN_POINT ( 'NONE',  ( -20.51205453730430506, -298.4240907695532883, -193.3606552284116447 ) ) ;
#30516=CARTESIAN_POINT ( 'NONE',  ( -37.52314650251574335, -287.1342226138090723, -345.9337310671166961 ) ) ;
#30517=CARTESIAN_POINT ( 'NONE',  ( 18.08959704142943536, -274.8196701557970982, -216.8395478004464394 ) ) ;
#30518=CARTESIAN_POINT ( 'NONE',  ( -55.43490633500003639, -293.7980920746240372, -197.9423173243462202 ) ) ;
#30519=CARTESIAN_POINT ( 'NONE',  ( 31.95455697924148097, -283.6233781216988064, -236.9535640164627637 ) ) ;
#30520=CARTESIAN_POINT ( 'NONE',  ( -109.6831941416651546, -276.2899097184970856, -290.7752472119889831 ) ) ;
#30522=CARTESIAN_POINT ( 'NONE',  ( -46.01834168528773006, -296.3437288632409263, -194.6567171476825706 ) ) ;
#30523=CARTESIAN_POINT ( 'NONE',  ( -7.473583189580038422, -275.9984385935695173, -337.0828405250173319 ) ) ;
#30524=CARTESIAN_POINT ( 'NONE',  ( -97.33699196483640037, -292.6655310050574030, -227.4814019588066287 ) ) ;
#30525=CARTESIAN_POINT ( 'NONE',  ( -67.91029542570618105, -292.5820101981540802, -203.7968353009282225 ) ) ;
#30526=CARTESIAN_POINT ( 'NONE',  ( -98.35515923680057426, -285.7359820032201014, -312.3470846972257391 ) ) ;
#30527=CARTESIAN_POINT ( 'NONE',  ( -7.437659946947347223, -293.8618978812461933, -200.0308022223674698 ) ) ;
#30528=CARTESIAN_POINT ( 'NONE',  ( 36.98493142505181197, -295.0962454731146067, -288.5502107766479867 ) ) ;
#30529=CARTESIAN_POINT ( 'NONE',  ( 33.11614360142508673, -293.6383040233006909, -289.5055582190390737 ) ) ;
#30530=CARTESIAN_POINT ( 'NONE',  ( 13.53060632349753512, -290.3405140215845108, -325.5407773122331605 ) ) ;
#30531=CARTESIAN_POINT ( 'NONE',  ( 26.72306369832012862, -282.2810918312300714, -313.0776960333909074 ) ) ;
#30532=CARTESIAN_POINT ( 'NONE',  ( -35.83875488410073729, -296.1506787407711272, -194.8015972003060483 ) ) ;
#30533=CARTESIAN_POINT ( 'NONE',  ( -107.9252799729639065, -284.7792795768385758, -239.4551215901402372 ) ) ;
#30534=CARTESIAN_POINT ( 'NONE',  ( -32.28449278934082400, -278.9680935930981036, -344.8855031816040082 ) ) ;
#30535=CARTESIAN_POINT ( 'NONE',  ( -67.69798870585597683, -284.4395894940728340, -203.5357766086774802 ) ) ;
#30536=CARTESIAN_POINT ( 'NONE',  ( 23.10682512407102962, -284.9465971018651089, -225.9654374940808736 ) ) ;
#30537=CARTESIAN_POINT ( 'NONE',  ( -110.8811787135462765, -276.9241037098828428, -252.0802173014898244 ) ) ;
#30540=CARTESIAN_POINT ( 'NONE',  ( -110.1576119294400655, -283.9809041161320238, -276.3470540060191638 ) ) ;
#30542=CARTESIAN_POINT ( 'NONE',  ( 24.79424682355846343, -283.3545586488428967, -315.1844259333581704 ) ) ;
#30543=CARTESIAN_POINT ( 'NONE',  ( -31.85559806373210989, -288.0434055663845925, -346.9819331810597873 ) ) ;
#30545=CARTESIAN_POINT ( 'NONE',  ( -74.92371665531206304, -279.1441543564675953, -336.6486164233569980 ) ) ;
#30546=CARTESIAN_POINT ( 'NONE',  ( -64.90168910481790476, -278.7197524321436504, -341.7875168366178400 ) ) ;
#30547=CARTESIAN_POINT ( 'NONE',  ( -22.19233475009214374, -280.0848186213743247, -198.8984997803549675 ) ) ;
#30548=CARTESIAN_POINT ( 'NONE',  ( 12.62934106623620778, -276.7323527833284516, -214.8411876572591268 ) ) ;
#30549=CARTESIAN_POINT ( 'NONE',  ( -13.96983070625157630, -284.3557710064802677, -199.2167885196802786 ) ) ;
#30551=CARTESIAN_POINT ( 'NONE',  ( -75.24784836585295977, -291.1488134150631595, -336.4637982716405418 ) ) ;
#30552=CARTESIAN_POINT ( 'NONE',  ( -10.38909202328236958, -293.6122944820573935, -338.5357686248896698 ) ) ;
#30554=CARTESIAN_POINT ( 'NONE',  ( 25.80882305186885972, -293.7217050023043612, -307.0230724968720892 ) ) ;
#30555=CARTESIAN_POINT ( 'NONE',  ( -113.3616278956509547, -291.7638138179833618, -259.8494096928264412 ) ) ;
#30556=CARTESIAN_POINT ( 'NONE',  ( 17.13324237519024962, -281.5070903846815895, -221.6130584558946168 ) ) ;
#30557=CARTESIAN_POINT ( 'NONE',  ( 98.51911204938808453, -298.6359351600565333, -193.6943702404669807 ) ) ;
#30558=CARTESIAN_POINT ( 'NONE',  ( 25.77280380391643888, -288.7858895839764273, -314.3828684735831303 ) ) ;
#30559=CARTESIAN_POINT ( 'NONE',  ( -34.66330532307965484, -289.3526358162238239, -347.2933641012310773 ) ) ;
#30560=CARTESIAN_POINT ( 'NONE',  ( -22.45967221883283216, -286.5811219193203669, -198.8206732889066473 ) ) ;
#30562=CARTESIAN_POINT ( 'NONE',  ( -96.13039596184697189, -238.4436301958426441, -339.9016185993384056 ) ) ;
#30563=CARTESIAN_POINT ( 'NONE',  ( -111.1601028361537118, -270.7551610738350973, -283.6484960496011922 ) ) ;
#30564=CARTESIAN_POINT ( 'NONE',  ( -78.73175922136113059, -276.8225119037208515, -330.7507890222076981 ) ) ;
#30565=CARTESIAN_POINT ( 'NONE',  ( -102.1365244259444296, -277.0073652384414231, -304.6518866663593599 ) ) ;
#30566=CARTESIAN_POINT ( 'NONE',  ( -85.79163217217676163, -273.0687217962955629, -210.5418202906136855 ) ) ;
#30567=CARTESIAN_POINT ( 'NONE',  ( -54.05466194891914000, -170.4008729781827469, -361.7658500053330499 ) ) ;
#30568=CARTESIAN_POINT ( 'NONE',  ( -51.23957477297972929, -275.9110914645577282, -345.5950687751796409 ) ) ;
#30569=CARTESIAN_POINT ( 'NONE',  ( 30.01459920551967642, -295.7720977988751656, -305.5335923264745475 ) ) ;
#30571=CARTESIAN_POINT ( 'NONE',  ( -30.80770831459367898, -292.6293228255084955, -197.5923376392886155 ) ) ;
#30572=CARTESIAN_POINT ( 'NONE',  ( -112.1195771238567289, -297.5765158148137743, -252.6854869237473622 ) ) ;
#30573=CARTESIAN_POINT ( 'NONE',  ( -34.57610967593285523, -287.7016389375725112, -343.8521342775541711 ) ) ;
#30574=CARTESIAN_POINT ( 'NONE',  ( -29.07414426903120486, -298.6454087753794511, -193.4219860267110391 ) ) ;
#30575=CARTESIAN_POINT ( 'NONE',  ( -110.3840863323154053, -296.7042681950358087, -271.4652349688109325 ) ) ;
#30579=CARTESIAN_POINT ( 'NONE',  ( -39.56976610098377733, -281.9445612293049521, -194.8211647523048384 ) ) ;
#30580=CARTESIAN_POINT ( 'NONE',  ( -81.48492659777620872, -280.5154970987184129, -211.7687278627689693 ) ) ;
#30581=CARTESIAN_POINT ( 'NONE',  ( -112.2414876114483349, -280.4745830070029911, -257.5550315501023988 ) ) ;
#30582=CARTESIAN_POINT ( 'NONE',  ( -76.92044237001688600, -271.9912772614846403, -208.1981795524608003 ) ) ;
#30583=CARTESIAN_POINT ( 'NONE',  ( 129.9467878515196162, -299.5541904835127980, -200.7046326357662167 ) ) ;
#30585=CARTESIAN_POINT ( 'NONE',  ( -3.150971852752717517, -280.6837172330894532, -205.8489241288082212 ) ) ;
#30586=CARTESIAN_POINT ( 'NONE',  ( 35.91178441532474608, -276.6471478528873718, -293.5577949579000006 ) ) ;
#30587=CARTESIAN_POINT ( 'NONE',  ( 7.077595747044981955, -278.4478500060455417, -330.8566067148845491 ) ) ;
#30588=CARTESIAN_POINT ( 'NONE',  ( -35.74218125625489506, -275.6072222886365921, -346.7681714343855219 ) ) ;
#30591=CARTESIAN_POINT ( 'NONE',  ( 34.05889703401961555, -283.8439620333300581, -294.6141347269443713 ) ) ;
#30592=CARTESIAN_POINT ( 'NONE',  ( -93.55736319168633486, -290.4123748477019262, -223.5184825260139689 ) ) ;
#30593=CARTESIAN_POINT ( 'NONE',  ( 37.27992447637554818, -286.6680819740904553, -251.7889364087348554 ) ) ;
#30595=CARTESIAN_POINT ( 'NONE',  ( -40.29695153435920929, -281.3296659843946372, -344.3154316117778535 ) ) ;
#30596=CARTESIAN_POINT ( 'NONE',  ( -91.18486269218223583, -282.4113280900047016, -320.5237411445754674 ) ) ;
#30597=CARTESIAN_POINT ( 'NONE',  ( 31.29889150567325018, -285.2513939124551143, -241.4215632714236790 ) ) ;
#30598=CARTESIAN_POINT ( 'NONE',  ( -4.181833166971558491, -281.7044770003787448, -204.8677379663166107 ) ) ;
#30600=CARTESIAN_POINT ( 'NONE',  ( 0.4536673384999292957, -280.9572038623820163, -336.5422734197180716 ) ) ;
#30601=CARTESIAN_POINT ( 'NONE',  ( 37.23450167266633315, -295.4439952157991911, -261.9249073331538398 ) ) ;
#30602=AXIS2_PLACEMENT_3D ( 'NONE', #30637, #59536, #32509 ) ;
#30603=CARTESIAN_POINT ( 'NONE',  ( -92.79855865534157999, -278.5264022390850300, -317.9891508070831492 ) ) ;
#30604=CARTESIAN_POINT ( 'NONE',  ( -40.75923848479533262, -288.0095491831267509, -195.2212290370152061 ) ) ;
#30607=CARTESIAN_POINT ( 'NONE',  ( -3.979611958363965307, -294.4088081039965346, -202.5509459563704695 ) ) ;
#30609=CARTESIAN_POINT ( 'NONE',  ( 37.58648830018066889, -273.4966165233839774, -266.0486861564917263 ) ) ;
#30610=CARTESIAN_POINT ( 'NONE',  ( -80.45847839062497542, -288.8171745226302392, -334.0265192067412272 ) ) ;
#30611=CARTESIAN_POINT ( 'NONE',  ( 33.88349486426316304, -292.2050873486961109, -289.7329880104829272 ) ) ;
#30613=CARTESIAN_POINT ( 'NONE',  ( -81.12651532718145120, -276.3461517254066280, -329.3876665403880111 ) ) ;
#30614=CARTESIAN_POINT ( 'NONE',  ( -86.90771506894039078, -295.4931450091982583, -215.0974260968129670 ) ) ;
#30615=CARTESIAN_POINT ( 'NONE',  ( -72.58070424613561045, -290.8442977220993839, -334.8549631737401455 ) ) ;
#30618=CARTESIAN_POINT ( 'NONE',  ( 19.87179139989343568, -291.3419617290406904, -219.8505388229311848 ) ) ;
#30619=CARTESIAN_POINT ( 'NONE',  ( 36.43062816853321095, -289.1968576723172077, -273.7767548167175278 ) ) ;
#30620=CARTESIAN_POINT ( 'NONE',  ( -90.06646705202767578, -289.5596800205086083, -215.5699902251751325 ) ) ;
#30622=CARTESIAN_POINT ( 'NONE',  ( -41.37321168113845715, -287.4257097674345118, -196.8698020162657087 ) ) ;
#30624=CARTESIAN_POINT ( 'NONE',  ( 17.00372509066372828, -287.6549784269396355, -221.3610290908781906 ) ) ;
#30625=CARTESIAN_POINT ( 'NONE',  ( 18.33188221679906249, -296.2381648642396499, -321.2196199662795948 ) ) ;
#30627=CARTESIAN_POINT ( 'NONE',  ( 2.984223698884188813, -289.7289947139753394, -335.5526725873778560 ) ) ;
#30628=CARTESIAN_POINT ( 'NONE',  ( -17.40241850694987846, -278.3283178353904646, -197.6917857409332839 ) ) ;
#30629=CARTESIAN_POINT ( 'NONE',  ( -100.4457392420967494, -278.3024794396129096, -314.4476753332854173 ) ) ;
#30631=CARTESIAN_POINT ( 'NONE',  ( 3.814254445228949297, -280.2563675923465780, -205.2448528453568599 ) ) ;
#30632=CARTESIAN_POINT ( 'NONE',  ( -89.28809463189834617, -299.2969937111515719, -216.6846486869660282 ) ) ;
#30633=CARTESIAN_POINT ( 'NONE',  ( -13.91783132143956081, -284.3557710075663749, -199.0583202572621815 ) ) ;
#30634=CARTESIAN_POINT ( 'NONE',  ( -110.8437467437025248, -273.8931351520964199, -270.3781919081613978 ) ) ;
#30635=CARTESIAN_POINT ( 'NONE',  ( 17.99918104428743604, -278.9956669220031813, -220.8813003536822634 ) ) ;
#30636=CARTESIAN_POINT ( 'NONE',  ( -95.63445920879816242, -281.9020240572296530, -317.5719306624231990 ) ) ;
#30637=CARTESIAN_POINT ( 'NONE',  ( 129.9467878515196162, -299.5541904835127980, -190.0176033293537898 ) ) ;
#30638=CARTESIAN_POINT ( 'NONE',  ( -12.11383863348450873, -275.2097445724068052, -342.4322470309236337 ) ) ;
#30639=CARTESIAN_POINT ( 'NONE',  ( -95.85124850480036685, -298.6968431830242707, -225.5371965432557033 ) ) ;
#30640=CARTESIAN_POINT ( 'NONE',  ( -114.0315902270491364, -283.4773981730751302, -269.9696266315025923 ) ) ;
#30641=CARTESIAN_POINT ( 'NONE',  ( -34.48036136891933978, -299.0300895859957109, -197.1253504873549787 ) ) ;
#30642=CARTESIAN_POINT ( 'NONE',  ( -107.5433937525821193, -274.3662323966685221, -240.0555830563437212 ) ) ;
#30643=CARTESIAN_POINT ( 'NONE',  ( 18.32177684422274666, -275.8906932691223233, -317.6227812859333426 ) ) ;
#30644=CARTESIAN_POINT ( 'NONE',  ( -56.28450734845745274, -297.2962361116501597, -342.9833174638788478 ) ) ;
#30645=CARTESIAN_POINT ( 'NONE',  ( -68.05192736183235525, -289.6110564114273416, -340.9718958268330198 ) ) ;
#30646=CARTESIAN_POINT ( 'NONE',  ( -8.071796992666712356, -278.5123757827599320, -200.6865678099490253 ) ) ;
#30647=CARTESIAN_POINT ( 'NONE',  ( -97.46223514609182814, -291.0299029512155471, -222.2516462156972352 ) ) ;
#30648=CARTESIAN_POINT ( 'NONE',  ( -95.96384920676541697, -288.9964934487360892, -314.2779737561940010 ) ) ;
#30649=CARTESIAN_POINT ( 'NONE',  ( 9.879838635458678908, -290.7018841847202566, -212.0265643798393853 ) ) ;
#30652=CARTESIAN_POINT ( 'NONE',  ( -101.7003222097025343, -289.5873346101069501, -305.0509993138333016 ) ) ;
#30654=CARTESIAN_POINT ( 'NONE',  ( -67.10891649974158213, -286.6125749206093474, -199.6028460789339078 ) ) ;
#30655=CARTESIAN_POINT ( 'NONE',  ( -105.5795714935544112, -292.8376638359844719, -285.9686137636504668 ) ) ;
#30656=CARTESIAN_POINT ( 'NONE',  ( 29.36425339623114183, -293.1069722472940953, -308.4570994373950725 ) ) ;
#30657=CARTESIAN_POINT ( 'NONE',  ( 31.95288522288795718, -283.2866210507178266, -302.9137357538254491 ) ) ;
#30658=CARTESIAN_POINT ( 'NONE',  ( -109.1926499096358754, -284.5565872633736717, -257.3896047553525932 ) ) ;
#30659=CARTESIAN_POINT ( 'NONE',  ( 15.96704342509009145, -277.5916653103729459, -320.9518418246126998 ) ) ;
#30660=CARTESIAN_POINT ( 'NONE',  ( 27.67942437163184266, -291.0802770493069147, -233.5935451657042279 ) ) ;
#30661=CARTESIAN_POINT ( 'NONE',  ( -63.43361009054868305, -272.4993633734621312, -201.7447627365557139 ) ) ;
#30663=CARTESIAN_POINT ( 'NONE',  ( 84.09003387609358526, 83.72762891241104910, -302.5758382668069544 ) ) ;
#30664=CARTESIAN_POINT ( 'NONE',  ( 13.37870584045069400, -294.0321486621642748, -328.3384794077394417 ) ) ;
#30665=CARTESIAN_POINT ( 'NONE',  ( -77.85284232898733592, -287.4239292079402617, -207.8486737744601385 ) ) ;
#30666=CARTESIAN_POINT ( 'NONE',  ( -113.0864293636219742, -297.7836666561045718, -258.2683156704083558 ) ) ;
#30667=CARTESIAN_POINT ( 'NONE',  ( -8.221955769621759558, -287.0952873052918903, -203.3093979678432390 ) ) ;
#30668=CARTESIAN_POINT ( 'NONE',  ( -107.3664055037144180, -277.2065017374494573, -301.9446155322348773 ) ) ;
#30669=CARTESIAN_POINT ( 'NONE',  ( 37.96039701746756378, -294.0075780040262430, -254.7111408871466267 ) ) ;
#30670=CARTESIAN_POINT ( 'NONE',  ( 38.12660995884635184, -285.5994405010960691, -263.0995957933824343 ) ) ;
#30671=CARTESIAN_POINT ( 'NONE',  ( 36.68266203864578046, -293.6200441925374776, -249.1911157424309522 ) ) ;
#30673=CARTESIAN_POINT ( 'NONE',  ( -89.83446885280095273, -291.6187172169491078, -219.6009296616121276 ) ) ;
#30677=CARTESIAN_POINT ( 'NONE',  ( 185.2856823004373155, 260.3293175955999459, -151.1391428731211874 ) ) ;
#30678=CARTESIAN_POINT ( 'NONE',  ( -64.32033406853761903, -287.2265360074954970, -198.9687809053639569 ) ) ;
#30679=CARTESIAN_POINT ( 'NONE',  ( -20.25526795762938548, -292.3380690714490129, -345.3683826091709648 ) ) ;
#30681=CARTESIAN_POINT ( 'NONE',  ( -48.38877429527233431, -282.1163982513141377, -342.8331003294917423 ) ) ;
#30682=CARTESIAN_POINT ( 'NONE',  ( -108.6384478555322914, -277.8501326739541923, -299.3872795430617657 ) ) ;
#30683=CARTESIAN_POINT ( 'NONE',  ( 19.00159051718811298, -284.2377290793045859, -319.6100979502661517 ) ) ;
#30684=CARTESIAN_POINT ( 'NONE',  ( -92.83366527638099797, -240.7103982912584286, -340.5308032049566691 ) ) ;
#30685=CARTESIAN_POINT ( 'NONE',  ( -68.95934043393330626, -282.0345319544100562, -339.9378496619090697 ) ) ;
#30686=CARTESIAN_POINT ( 'NONE',  ( -35.87645741426449320, -284.0907313453803908, -195.7306961024721943 ) ) ;
#30688=CARTESIAN_POINT ( 'NONE',  ( 17.18393258882466412, -276.6797861019121001, -217.6810709008790070 ) ) ;
#30689=CARTESIAN_POINT ( 'NONE',  ( -86.14604871652491624, -297.8455293533723989, -215.9908687615359497 ) ) ;
#30690=CARTESIAN_POINT ( 'NONE',  ( -50.57634116159846371, -293.9095417438324489, -342.6528032128883865 ) ) ;
#30691=CARTESIAN_POINT ( 'NONE',  ( -111.6347024013553408, -279.4529540461732608, -250.4642884469988076 ) ) ;
#30692=CARTESIAN_POINT ( 'NONE',  ( -16.38086886027196698, -276.7737087032643331, -340.3401131848896171 ) ) ;
#30693=CARTESIAN_POINT ( 'NONE',  ( -114.0330990441454873, -273.6675114159231157, -267.5188803404774376 ) ) ;
#30694=CARTESIAN_POINT ( 'NONE',  ( -14.69415164179740252, -275.6858307667873760, -343.6873177583000256 ) ) ;
#30695=CARTESIAN_POINT ( 'NONE',  ( -104.6885212946842927, -255.7827803519188592, -326.5688778022348515 ) ) ;
#30696=CARTESIAN_POINT ( 'NONE',  ( -93.00135176084691579, -275.8510104536460403, -320.6493964774192023 ) ) ;
#30699=CARTESIAN_POINT ( 'NONE',  ( -101.0683720381171184, -298.5365188988735099, -228.1766677701635331 ) ) ;
#30701=DIRECTION ( 'NONE',  ( 0.000000000000000000, 0.000000000000000000, -1.000000000000000000 ) ) ;
#30702=CARTESIAN_POINT ( 'NONE',  ( -48.36163832974614252, -284.2753933237065667, -342.8372315302723905 ) ) ;
#30703=CARTESIAN_POINT ( 'NONE',  ( -112.1354564836506995, -286.1386677393974765, -284.0610391722537997 ) ) ;
#30704=CARTESIAN_POINT ( 'NONE',  ( -37.27245837176452881, -285.4015903195714827, -197.2467616316953354 ) ) ;
#30705=CARTESIAN_POINT ( 'NONE',  ( -110.9551997794928013, -277.0204358685767261, -265.1177333231860302 ) ) ;
#30706=CARTESIAN_POINT ( 'NONE',  ( -96.07948831425808578, -285.7837963392622100, -315.7772094309784165 ) ) ;
#30707=CARTESIAN_POINT ( 'NONE',  ( -102.7625571579186214, -277.4903772484469755, -236.3263874081253277 ) ) ;
#30708=CARTESIAN_POINT ( 'NONE',  ( -51.32644489812637545, -278.3148633365489673, -342.3239763638684963 ) ) ;
#30710=CARTESIAN_POINT ( 'NONE',  ( -16.62921603255674796, -274.8192962103832997, -200.2442429511368687 ) ) ;
#30711=CARTESIAN_POINT ( 'NONE',  ( 39.11851154794064911, -282.4568750517863123, -278.4912598217030677 ) ) ;
#30712=VECTOR ( 'NONE', #79226, 1000.000000000000000 ) ;
#30713=CARTESIAN_POINT ( 'NONE',  ( 21.56694273956899366, -282.7113922162508288, -319.8515079481271073 ) ) ;
#30717=CARTESIAN_POINT ( 'NONE',  ( 13.40174600858478904, -288.6132600908331369, -214.0287920440416372 ) ) ;
#30718=CARTESIAN_POINT ( 'NONE',  ( -49.97176851101051653, -297.0840217217794930, -198.2980685109567105 ) ) ;
#30719=CARTESIAN_POINT ( 'NONE',  ( 20.30777971561858308, -292.2105301521623346, -219.4506501077159442 ) ) ;
#30721=CARTESIAN_POINT ( 'NONE',  ( 8.395258187434462727, -286.8926716278811568, -328.1438004621078903 ) ) ;
#30722=CARTESIAN_POINT ( 'NONE',  ( -66.57970414856659147, -288.0173736524386641, -337.9471555936756886 ) ) ;
#30723=CARTESIAN_POINT ( 'NONE',  ( 17.17531811845548262, -288.0571566266493733, -221.1994534386860494 ) ) ;
#30724=CARTESIAN_POINT ( 'NONE',  ( -97.22240257946876341, -275.9343644740023933, -315.5408375941399868 ) ) ;
#30725=CARTESIAN_POINT ( 'NONE',  ( 5.094724261253341879, -286.8885627266888037, -333.6508509495091630 ) ) ;
#30726=CARTESIAN_POINT ( 'NONE',  ( -49.05808743230583246, -287.9031698768554293, -196.2295824839782483 ) ) ;
#30727=CARTESIAN_POINT ( 'NONE',  ( 6.835931173569454344, -286.4529149437168485, -331.2394755736891625 ) ) ;
#30728=CARTESIAN_POINT ( 'NONE',  ( 33.18927607508316413, -282.7531795207079881, -290.0788725295082600 ) ) ;
#30729=CARTESIAN_POINT ( 'NONE',  ( -67.61434734465515817, -293.6560919866633412, -201.5459623180830988 ) ) ;
#30732=CARTESIAN_POINT ( 'NONE',  ( -110.1969538447277870, -298.2165402983124523, -290.3967414035506636 ) ) ;
#30733=CARTESIAN_POINT ( 'NONE',  ( 11.42103552357760066, -279.9463758745067139, -215.8194152378700608 ) ) ;
#30734=CARTESIAN_POINT ( 'NONE',  ( 30.80017799712559778, -279.1391369788243537, -238.9047102129392499 ) ) ;
#30735=CARTESIAN_POINT ( 'NONE',  ( 39.28081183249745578, -292.6771637971945097, -264.6035593893051896 ) ) ;
#30736=CARTESIAN_POINT ( 'NONE',  ( -39.16791977715406858, -296.4287598082912041, -196.5711688138334807 ) ) ;
#30737=CARTESIAN_POINT ( 'NONE',  ( 36.53205513495402101, -273.7558504733202085, -279.9353271203199256 ) ) ;
#30738=CARTESIAN_POINT ( 'NONE',  ( -72.34480413197637461, -296.8407151454754285, -334.9976621723017161 ) ) ;
#30739=CARTESIAN_POINT ( 'NONE',  ( -46.03152702926329454, -296.4237223872028721, -194.5508636611600082 ) ) ;
#30740=CARTESIAN_POINT ( 'NONE',  ( -107.4489023662299871, -294.4127390446410004, -299.8053167439474578 ) ) ;
#30741=AXIS2_PLACEMENT_3D ( 'NONE', #48649, #77549, #41540 ) ;
#30743=CARTESIAN_POINT ( 'NONE',  ( 36.12165325131429938, -294.9106460289418123, -265.2575402751756428 ) ) ;
#30745=CARTESIAN_POINT ( 'NONE',  ( -2.371225574760046584, -293.3302217590810415, -206.0844021007544598 ) ) ;
#30748=CARTESIAN_POINT ( 'NONE',  ( -84.46430106641275870, -283.4271193461231633, -211.5574847568799441 ) ) ;
#30749=CARTESIAN_POINT ( 'NONE',  ( -94.77343848336226984, -295.9167239171960091, -315.4232465329353658 ) ) ;
#30751=CARTESIAN_POINT ( 'NONE',  ( -114.3548908130070174, -284.5210348520636785, -272.8492333268528682 ) ) ;
#30752=CARTESIAN_POINT ( 'NONE',  ( -35.39804502326355617, -281.9964866374365897, -194.8132253889213814 ) ) ;
#30753=CARTESIAN_POINT ( 'NONE',  ( -12.70645810459626368, -286.0305970408420535, -197.4306775484280649 ) ) ;
#30754=CARTESIAN_POINT ( 'NONE',  ( -110.4975654402052356, -288.7547481693756026, -254.6052365074582440 ) ) ;
#30755=CARTESIAN_POINT ( 'NONE',  ( -95.95921662488163406, -270.6952119285918457, -223.5744983911110353 ) ) ;
#30757=CARTESIAN_POINT ( 'NONE',  ( -73.78572110730844713, -284.2422806971239879, -206.5258643163653574 ) ) ;
#30758=CARTESIAN_POINT ( 'NONE',  ( -113.3578563845434246, -289.6048192971995832, -259.8221587332401441 ) ) ;
#30760=CARTESIAN_POINT ( 'NONE',  ( 14.89679763691791514, -295.9012026312825014, -322.5634038923562343 ) ) ;
#30761=CARTESIAN_POINT ( 'NONE',  ( -98.96352418531954243, -280.5823069761846682, -225.1576488086723202 ) ) ;
#30762=CARTESIAN_POINT ( 'NONE',  ( -50.21194661902687528, -293.2356056660836430, -344.6618997651258383 ) ) ;
#30763=CARTESIAN_POINT ( 'NONE',  ( 9.293302485419381753, -280.3800044079196709, -214.1056646280910343 ) ) ;
#30764=CARTESIAN_POINT ( 'NONE',  ( -70.80595324782682098, -295.6480367922205801, -339.7236182855646689 ) ) ;
#30766=CARTESIAN_POINT ( 'NONE',  ( -112.1767626617573939, -282.4942027894425109, -281.1731583314693808 ) ) ;
#30768=CARTESIAN_POINT ( 'NONE',  ( -50.61145333056632012, -281.8828257199812697, -196.5443563635312785 ) ) ;
#30769=CARTESIAN_POINT ( 'NONE',  ( -39.70861269458068676, -294.1413156074694371, -343.5706249872390003 ) ) ;
#30770=CARTESIAN_POINT ( 'NONE',  ( 17.58432135626699022, -296.7395371843010707, -195.3798368471506706 ) ) ;
#30774=CARTESIAN_POINT ( 'NONE',  ( -6.103590747113877057, -282.4445556861036266, -202.5531599629256050 ) ) ;
#30775=CARTESIAN_POINT ( 'NONE',  ( -80.19593387614979463, -295.1579863652195854, -329.5346178904471799 ) ) ;
#30777=CARTESIAN_POINT ( 'NONE',  ( 10.64812456238590777, -278.1952119285918457, -210.2361428286349110 ) ) ;
#30778=CARTESIAN_POINT ( 'NONE',  ( -85.69866662021578918, -272.5992459651270678, -210.6471111527235678 ) ) ;
#30779=CARTESIAN_POINT ( 'NONE',  ( -34.66718048847827305, -290.3343699242483353, -346.8212070397212869 ) ) ;
#30780=CARTESIAN_POINT ( 'NONE',  ( -102.4086035363959724, -290.8362989218113626, -237.1539389000297149 ) ) ;
#30781=CARTESIAN_POINT ( 'NONE',  ( -14.10847418865916936, -281.8790414658838586, -200.3720279850016368 ) ) ;
#30782=CARTESIAN_POINT ( 'NONE',  ( 16.01120344943208451, -276.4240061499760372, -219.2978712780624733 ) ) ;
#30784=CARTESIAN_POINT ( 'NONE',  ( -81.51468190424904492, -278.2311176008949474, -211.6809444703450822 ) ) ;
#30785=CARTESIAN_POINT ( 'NONE',  ( 27.10686732003000898, -278.0655883576399106, -308.7197258924548464 ) ) ;
#30787=CARTESIAN_POINT ( 'NONE',  ( 13.96605773749421431, -274.5817538268141789, -212.8745875764777793 ) ) ;
#30788=CARTESIAN_POINT ( 'NONE',  ( -93.66169169272090755, -293.1524323693145107, -221.6849148624908707 ) ) ;
#30791=CARTESIAN_POINT ( 'NONE',  ( -19.65180315312841586, -290.4167113165010505, -196.6364640528616121 ) ) ;
#30792=CARTESIAN_POINT ( 'NONE',  ( -75.21798337578533733, -297.1992919624360070, -207.8727383157991824 ) ) ;
#30794=CARTESIAN_POINT ( 'NONE',  ( -2.390813492799769957, -294.0261305994960139, -202.5147473267676901 ) ) ;
#30795=CARTESIAN_POINT ( 'NONE',  ( -85.28047601435908120, -286.1948066931273615, -330.5268031993605859 ) ) ;
#30796=CARTESIAN_POINT ( 'NONE',  ( 37.46379743484509106, -289.5968253763476810, -273.8197834064524159 ) ) ;
#30797=CARTESIAN_POINT ( 'NONE',  ( -6.781697966510144227, -274.6499094321674193, -338.6700829691203580 ) ) ;
#30798=CARTESIAN_POINT ( 'NONE',  ( 24.22992037913066099, -276.9014550049094510, -228.5022783285045307 ) ) ;
#30799=CARTESIAN_POINT ( 'NONE',  ( -58.03218868781078754, -289.8627521962294509, -198.8004353172029539 ) ) ;
#30800=CARTESIAN_POINT ( 'NONE',  ( -40.97327799142219362, -281.8673538163822059, -194.6704154582403987 ) ) ;
#30801=ORIENTED_EDGE ( 'NONE', *, *, #57401, .F. ) ;
#30802=CARTESIAN_POINT ( 'NONE',  ( -42.94900150372097869, -282.4732346736718114, -343.2978358253071178 ) ) ;
#30803=CARTESIAN_POINT ( 'NONE',  ( -110.3680817387783009, -279.3341855749993670, -293.9550698515365070 ) ) ;
#30805=CARTESIAN_POINT ( 'NONE',  ( -52.85229397362792270, -282.0414629774623450, -345.4315308849867279 ) ) ;
#30806=CARTESIAN_POINT ( 'NONE',  ( -1.566724959004111906, -277.5308946173458935, -338.2799766684636324 ) ) ;
#30808=CARTESIAN_POINT ( 'NONE',  ( 7.846202039818450658, -277.9678887343407041, -331.9144443956383839 ) ) ;
#30809=CARTESIAN_POINT ( 'NONE',  ( 27.33386217378599881, -283.6233781216987495, -239.1787733560258573 ) ) ;
#30812=CARTESIAN_POINT ( 'NONE',  ( -101.8747147855665105, -298.0399770324070232, -308.6796865119803783 ) ) ;
#30814=CARTESIAN_POINT ( 'NONE',  ( -21.04731783917208787, -289.9177925857937339, -341.8364226580233094 ) ) ;
#30815=CARTESIAN_POINT ( 'NONE',  ( -64.96475342421375387, -275.4347424554158579, -339.7616297575960402 ) ) ;
#30816=CARTESIAN_POINT ( 'NONE',  ( -95.59952814923676101, -291.6467394332894401, -319.1665308045383540 ) ) ;
#30817=CARTESIAN_POINT ( 'NONE',  ( -95.18997482794893017, -290.5291158257365964, -225.6680560737433723 ) ) ;
#30818=CARTESIAN_POINT ( 'NONE',  ( 12.37128700372701573, -287.8887207784222824, -329.0820325998622593 ) ) ;
#30820=CARTESIAN_POINT ( 'NONE',  ( -109.7094852617887994, -283.1408187200852353, -255.8923899166755120 ) ) ;
#30821=CARTESIAN_POINT ( 'NONE',  ( -66.79771287259356427, -291.3025309230109201, -338.5571333640543799 ) ) ;
#30822=CARTESIAN_POINT ( 'NONE',  ( -95.49234025866557829, -283.6641016190898767, -225.0724244462670924 ) ) ;
#30823=CARTESIAN_POINT ( 'NONE',  ( 35.63151381142870378, -282.9871202483654429, -279.5030732748415403 ) ) ;
#30824=CARTESIAN_POINT ( 'NONE',  ( 25.66546950460050880, -289.0756815752255307, -314.3034804150059927 ) ) ;
#30826=CARTESIAN_POINT ( 'NONE',  ( -108.0337153144891005, -279.2885519241328893, -251.8558646779087553 ) ) ;
#30827=CARTESIAN_POINT ( 'NONE',  ( 1.512008411810999542, -291.3538862561458700, -204.2823279412429827 ) ) ;
#30828=CARTESIAN_POINT ( 'NONE',  ( 11.96611122471376731, -287.5199487840773713, -211.3603920930030995 ) ) ;
#30829=CARTESIAN_POINT ( 'NONE',  ( 22.36136238827849354, -288.6962779021726533, -318.9109306136004989 ) ) ;
#30830=CARTESIAN_POINT ( 'NONE',  ( -108.4248121873693691, -284.4989454371670377, -287.0347275724043925 ) ) ;
#30833=CARTESIAN_POINT ( 'NONE',  ( 22.12362110497789658, -294.7741227646307607, -223.3916887767994979 ) ) ;
#30835=CARTESIAN_POINT ( 'NONE',  ( 37.86934828177489720, -292.4143589055810253, -284.4531096408489361 ) ) ;
#30837=CARTESIAN_POINT ( 'NONE',  ( -51.33755177823420013, -276.2942651994949301, -342.2466143222532651 ) ) ;
#30838=CARTESIAN_POINT ( 'NONE',  ( -110.7133623401958999, -296.1923658369367445, -247.1648483659918440 ) ) ;
#30840=CARTESIAN_POINT ( 'NONE',  ( 30.50154763801040758, -291.6477892382942514, -241.4554683993791286 ) ) ;
#30841=CARTESIAN_POINT ( 'NONE',  ( -73.32013459407018274, -295.8078636147137104, -205.6809334755501197 ) ) ;
#30842=CARTESIAN_POINT ( 'NONE',  ( -77.48509179236710054, -292.7052443709765157, -208.9148926311063690 ) ) ;
#30843=CARTESIAN_POINT ( 'NONE',  ( 36.01738309023951246, -294.6369107577861541, -270.7478900384898566 ) ) ;
#30846=CARTESIAN_POINT ( 'NONE',  ( 18.15839412620846716, -292.2587546078964920, -321.1297799080661548 ) ) ;
#30847=CARTESIAN_POINT ( 'NONE',  ( -99.40254063079866853, -299.1233527197991293, -228.1588794409857428 ) ) ;
#30848=CARTESIAN_POINT ( 'NONE',  ( 35.50722417909328499, -288.3946207428232356, -262.8482839552062273 ) ) ;
#30849=CARTESIAN_POINT ( 'NONE',  ( -4.684356370965116589, -278.6040342858181589, -338.2863156209719477 ) ) ;
#30850=CARTESIAN_POINT ( 'NONE',  ( -113.2257384258998201, -277.3646709480278787, -260.2165416380571514 ) ) ;
#30852=CARTESIAN_POINT ( 'NONE',  ( -112.3420280466402517, -272.1133616190666089, -253.3827906410119226 ) ) ;
#30853=CARTESIAN_POINT ( 'NONE',  ( 10.82214414349227560, -280.4603475647468258, -327.1876582976967143 ) ) ;
#30854=CARTESIAN_POINT ( 'NONE',  ( -74.59880919751368822, -277.9648036321973450, -203.8904609995308874 ) ) ;
#30855=CARTESIAN_POINT ( 'NONE',  ( -109.8521900102618218, -295.0800244483023675, -282.3391117895540106 ) ) ;
#30856=DIRECTION ( 'NONE',  ( 0.000000000000000000, 0.000000000000000000, 1.000000000000000000 ) ) ;
#30857=CARTESIAN_POINT ( 'NONE',  ( 34.72474627639046219, -276.0410783374624657, -258.0263121627884857 ) ) ;
#30859=CARTESIAN_POINT ( 'NONE',  ( -105.7563170623370326, -288.9866227387603885, -238.6481710770466123 ) ) ;
#30860=CARTESIAN_POINT ( 'NONE',  ( -97.29007649960774984, -289.9041391513514441, -318.7057374775315566 ) ) ;
#30861=CARTESIAN_POINT ( 'NONE',  ( -19.02205139238770215, -276.2874411217178476, -197.4073416543744486 ) ) ;
#30862=CARTESIAN_POINT ( 'NONE',  ( -112.0408566726942183, -294.6096294032310539, -265.8817837155626194 ) ) ;
#30863=CARTESIAN_POINT ( 'NONE',  ( 0.7793460100420999126, -281.7543709765553785, -337.0917176694905493 ) ) ;
#30865=CARTESIAN_POINT ( 'NONE',  ( 15.69617743849259917, -280.3017984011779618, -323.4610907491652370 ) ) ;
#30867=CARTESIAN_POINT ( 'NONE',  ( -109.6653655975623565, -289.5149669882046624, -257.5645647395224955 ) ) ;
#30868=CARTESIAN_POINT ( 'NONE',  ( -107.3463383787781993, -282.3666718629504544, -295.2168867701692534 ) ) ;
#30871=CARTESIAN_POINT ( 'NONE',  ( 21.77464982989269160, -290.9185876728425342, -224.1856021271876216 ) ) ;
#30872=CARTESIAN_POINT ( 'NONE',  ( -89.63850011275077634, -279.4044360939305989, -322.5055873775744999 ) ) ;
#30873=CARTESIAN_POINT ( 'NONE',  ( 19.49924152228387442, -283.4588150744407358, -321.7916005121845728 ) ) ;
#30874=CARTESIAN_POINT ( 'NONE',  ( 15.04657443394469851, -272.8641938875279607, -215.9112981046183108 ) ) ;
#30875=CARTESIAN_POINT ( 'NONE',  ( -37.28087273214584485, -286.0528980263154040, -197.3487048133511053 ) ) ;
#30876=CARTESIAN_POINT ( 'NONE',  ( 25.89107511748261814, -277.4907927886520724, -308.0040595643965844 ) ) ;
#30877=CARTESIAN_POINT ( 'NONE',  ( 9.775828408964978067, -277.1865735196354876, -326.3302186632087114 ) ) ;
#30879=CARTESIAN_POINT ( 'NONE',  ( -90.50377291779354039, -287.2993055973473702, -217.4574823376597124 ) ) ;
#30882=CARTESIAN_POINT ( 'NONE',  ( -113.1387418114993437, -296.5550293662739136, -256.8035195019820662 ) ) ;
#30883=CARTESIAN_POINT ( 'NONE',  ( 10.05590126678781893, -288.6891379060571126, -212.6955807735517681 ) ) ;
#30885=CARTESIAN_POINT ( 'NONE',  ( 13.79469577742117181, -285.9094976428776249, -334.5364918783848793 ) ) ;
#30886=CARTESIAN_POINT ( 'NONE',  ( -112.9294888653194704, -277.6352290505569158, -257.4004581242679137 ) ) ;
#30887=CARTESIAN_POINT ( 'NONE',  ( -34.96473907088594757, -290.4813829905241960, -194.1851841416402351 ) ) ;
#30888=AXIS2_PLACEMENT_3D ( 'NONE', #46326, #67665, #82325 ) ;
#30889=CARTESIAN_POINT ( 'NONE',  ( -109.0445793503759262, -286.2952361977594364, -253.2948059606713969 ) ) ;
#30890=CARTESIAN_POINT ( 'NONE',  ( -111.3653967849307236, -280.3443673796571716, -267.8965756014687827 ) ) ;
#30891=CARTESIAN_POINT ( 'NONE',  ( 31.16723846048784807, -289.4169750666260938, -304.3202993333458153 ) ) ;
#30892=CARTESIAN_POINT ( 'NONE',  ( 36.68151218948661096, -283.7072261756798639, -282.4261371738191997 ) ) ;
#30893=CARTESIAN_POINT ( 'NONE',  ( 26.06808917318163310, -276.2965745335932297, -314.1363398641886420 ) ) ;
#30894=CARTESIAN_POINT ( 'NONE',  ( -40.56430231468502257, -296.0315640567754372, -195.7730783687483722 ) ) ;
#30895=CARTESIAN_POINT ( 'NONE',  ( -72.50491866364795612, -279.4330608981057367, -201.8442911778038820 ) ) ;
#30897=CARTESIAN_POINT ( 'NONE',  ( -110.6990019307856983, -298.6359535463627140, -257.7111981572658692 ) ) ;
#30900=CARTESIAN_POINT ( 'NONE',  ( 10.59707575819634329, -283.1948066931273047, -210.1954327657594490 ) ) ;
#30901=CARTESIAN_POINT ( 'NONE',  ( -75.89895036840451326, -271.7849774771071907, -204.8227570746032882 ) ) ;
#30903=CARTESIAN_POINT ( 'NONE',  ( -56.62244419163911147, -276.8150031597948555, -340.8852257245467285 ) ) ;
#30905=CARTESIAN_POINT ( 'NONE',  ( -71.24096313766156641, -274.8196076151936040, -201.6672413429360518 ) ) ;
#30906=CARTESIAN_POINT ( 'NONE',  ( 24.40962406065657575, -280.0030237770741337, -224.7585503524113619 ) ) ;
#30907=CARTESIAN_POINT ( 'NONE',  ( -50.91561475274457393, -290.9879667829274581, -343.1714857444937934 ) ) ;
#30908=CARTESIAN_POINT ( 'NONE',  ( -65.30611237074187159, -299.2134579309066567, -199.3067523476892404 ) ) ;
#30909=CARTESIAN_POINT ( 'NONE',  ( -46.09978616359826020, -299.1484808340330801, -194.2604961254596105 ) ) ;
#30910=CARTESIAN_POINT ( 'NONE',  ( -52.77206598574392871, -293.8542785152798160, -197.0826938709160743 ) ) ;
#30911=CARTESIAN_POINT ( 'NONE',  ( 2.045116585425529099, -280.5238692333006725, -334.0510667200915691 ) ) ;
#30912=CARTESIAN_POINT ( 'NONE',  ( 19.03950347069537585, -282.7932157371956805, -221.7362703742093402 ) ) ;
#30913=CARTESIAN_POINT ( 'NONE',  ( 0.3045703254873016741, -272.5762476158075742, -205.8899693141657963 ) ) ;
#30914=CARTESIAN_POINT ( 'NONE',  ( -113.4083212519305448, -286.0850304614825745, -275.6824285141259452 ) ) ;
#30916=CARTESIAN_POINT ( 'NONE',  ( -82.74845060867620816, -288.6102892066414256, -327.9150325620414037 ) ) ;
#30917=CARTESIAN_POINT ( 'NONE',  ( 198.8200449370011995, 284.3224334190195464, -111.7342436523391029 ) ) ;
#30919=CARTESIAN_POINT ( 'NONE',  ( 17.83872032041365685, -287.9009263383961184, -318.2615888902410575 ) ) ;
#30921=CARTESIAN_POINT ( 'NONE',  ( -67.74610994585918888, -284.5215885327106662, -340.7675408007664828 ) ) ;
#30922=CARTESIAN_POINT ( 'NONE',  ( 34.14117166887788812, -275.6880084067138910, -255.3908159382060603 ) ) ;
#30923=CARTESIAN_POINT ( 'NONE',  ( -104.3332548732852700, -289.9584105575837043, -233.0298428661952244 ) ) ;
#30924=CARTESIAN_POINT ( 'NONE',  ( 22.44925252602147481, -282.8530277955014185, -318.7384346170857157 ) ) ;
#30925=CARTESIAN_POINT ( 'NONE',  ( 16.71812759666127590, -282.3241927860921692, -216.4331443942766953 ) ) ;
#30926=CARTESIAN_POINT ( 'NONE',  ( -79.14468289328844719, -283.9329756154883171, -335.0005403454044313 ) ) ;
#30927=CARTESIAN_POINT ( 'NONE',  ( -83.43773839673744419, -279.3999851422124721, -213.6904333508806531 ) ) ;
#30928=CARTESIAN_POINT ( 'NONE',  ( -4.771743288812454686, -271.9809262143061233, -202.8022627189028810 ) ) ;
#30929=CARTESIAN_POINT ( 'NONE',  ( 174.5893627881048928, 243.1951182970949503, -179.8094511266240829 ) ) ;
#30931=CARTESIAN_POINT ( 'NONE',  ( -10.57508152806877355, -278.7023282806881639, -340.2437092007280626 ) ) ;
#30932=CARTESIAN_POINT ( 'NONE',  ( 64.01848135404819118, 48.19560674472151618, -318.4631135849222119 ) ) ;
#30933=CARTESIAN_POINT ( 'NONE',  ( -96.17743270066428352, -296.5081959115459540, -226.9550913852802125 ) ) ;
#30934=CARTESIAN_POINT ( 'NONE',  ( 20.33671706934794798, -292.3695704743377064, -219.4223832503387825 ) ) ;
#30935=CARTESIAN_POINT ( 'NONE',  ( 168.2916594723880905, 229.6308326061414391, -190.1149449454625824 ) ) ;
#30937=CARTESIAN_POINT ( 'NONE',  ( -112.5801950777285185, -271.4151616006713539, -256.2053483126125570 ) ) ;
#30938=CARTESIAN_POINT ( 'NONE',  ( -61.53631049351803028, -287.7716523653417653, -340.0824292416541539 ) ) ;
#30939=CARTESIAN_POINT ( 'NONE',  ( -89.35060544490218604, -297.6538926294820726, -323.4044528949978030 ) ) ;
#30941=CARTESIAN_POINT ( 'NONE',  ( -17.05169117012472668, -287.6347035934186920, -199.6711062099155356 ) ) ;
#30942=VERTEX_POINT ( 'NONE', #16380 ) ;
#30943=CARTESIAN_POINT ( 'NONE',  ( 23.84869874287717195, -295.1128094497666439, -316.7136292387993421 ) ) ;
#30944=CARTESIAN_POINT ( 'NONE',  ( -76.15450780505386774, -284.0781456425465876, -332.3204980065190171 ) ) ;
#30945=CARTESIAN_POINT ( 'NONE',  ( -113.5539487023561094, -271.5799049758838919, -261.8062552366379805 ) ) ;
#30946=CARTESIAN_POINT ( 'NONE',  ( 26.35330516716049942, -293.7864222017060456, -227.2895773231536225 ) ) ;
#30947=CARTESIAN_POINT ( 'NONE',  ( 22.24296058536637943, -294.6985700973331745, -319.0561808675521434 ) ) ;
#30948=CARTESIAN_POINT ( 'NONE',  ( -85.93061022477877486, -291.5235007570179278, -215.8126428492608966 ) ) ;
#30951=CARTESIAN_POINT ( 'NONE',  ( -34.83466128549527241, -299.9436287636900147, -194.5955260062804939 ) ) ;
#30952=CARTESIAN_POINT ( 'NONE',  ( 15.76287283857926269, -273.5791570138986231, -215.1532105064771656 ) ) ;
#30955=CARTESIAN_POINT ( 'NONE',  ( -35.71909818086986377, -276.5399964837521338, -347.2955810091828539 ) ) ;
#30956=CARTESIAN_POINT ( 'NONE',  ( -67.36449829597728467, -272.0515927815287114, -202.9301278194689075 ) ) ;
#30957=CARTESIAN_POINT ( 'NONE',  ( -105.5867528592758191, -280.7984783900357115, -241.1467678195408553 ) ) ;
#30958=CARTESIAN_POINT ( 'NONE',  ( -26.87030663151578480, -275.0571566278396745, -343.8540795280833322 ) ) ;
#30959=CARTESIAN_POINT ( 'NONE',  ( -104.0860325928904189, -298.1682404018121133, -239.7047398712782922 ) ) ;
#30960=CARTESIAN_POINT ( 'NONE',  ( -67.16426205753275269, -274.5925621974017190, -203.4592398691484618 ) ) ;
#30961=CARTESIAN_POINT ( 'NONE',  ( -80.69093503821387969, -275.2335496103571018, -207.8888690576729914 ) ) ;
#30962=CARTESIAN_POINT ( 'NONE',  ( -16.21382576296086242, -272.3439297494500124, -197.9742533303364951 ) ) ;
#30963=CARTESIAN_POINT ( 'NONE',  ( 33.54693810343505334, -294.4388429849327622, -288.2131105377094968 ) ) ;
#30964=CARTESIAN_POINT ( 'NONE',  ( -33.45934403757850362, -290.6766683638933841, -196.8617764458852832 ) ) ;
#30966=CARTESIAN_POINT ( 'NONE',  ( -28.60179523275668600, -277.4366107036450444, -346.8550915018040541 ) ) ;
#30967=CARTESIAN_POINT ( 'NONE',  ( -32.69315238843643101, -274.2790156907939831, -197.4967488178583892 ) ) ;
#30968=CARTESIAN_POINT ( 'NONE',  ( -101.0180605870684900, -282.6741351852214734, -312.8663388961496139 ) ) ;
#30969=CARTESIAN_POINT ( 'NONE',  ( -36.27430838535670432, -297.0389920590856718, -345.5330013424953108 ) ) ;
#30971=CARTESIAN_POINT ( 'NONE',  ( -11.95638942263939875, -285.5883862540134146, -201.7448828240623016 ) ) ;
#30973=CARTESIAN_POINT ( 'NONE',  ( -31.79754602902082183, -280.9821973046804828, -345.3359988806927845 ) ) ;
#30974=CARTESIAN_POINT ( 'NONE',  ( -0.9918388780831031148, -274.8028678399028877, -334.8912821822397632 ) ) ;
#30975=CARTESIAN_POINT ( 'NONE',  ( 7.928702925703531967, -274.9947406118189974, -328.4429786278427628 ) ) ;
#30976=CARTESIAN_POINT ( 'NONE',  ( 37.62044297025344974, -283.5992433719841301, -274.0158655108357948 ) ) ;
#30977=CARTESIAN_POINT ( 'NONE',  ( 34.76071216147933995, -276.5771566678704403, -256.6362264438267289 ) ) ;
#30979=CARTESIAN_POINT ( 'NONE',  ( -29.89656310287272234, -272.5447819910657472, -194.5257017870235927 ) ) ;
#30981=CARTESIAN_POINT ( 'NONE',  ( -22.94293154858993589, -282.2359772141625740, -196.5334739464187237 ) ) ;
#30983=CARTESIAN_POINT ( 'NONE',  ( 15.27851364362460274, -288.7085948671503957, -216.1354109878155327 ) ) ;
#30985=CARTESIAN_POINT ( 'NONE',  ( -65.11036602495053671, -287.4146716371830053, -340.0853651668093676 ) ) ;
#30988=CARTESIAN_POINT ( 'NONE',  ( -68.20055119649290987, -296.4325544396785403, -203.7526220073208663 ) ) ;
#30989=CARTESIAN_POINT ( 'NONE',  ( -92.57663154455117649, -289.3899842749509617, -220.7440493597310933 ) ) ;
#30990=CARTESIAN_POINT ( 'NONE',  ( -75.88346903603265048, -208.4961600436150491, -353.2410745688453062 ) ) ;
#30991=CARTESIAN_POINT ( 'NONE',  ( -47.51962034187837247, -295.9227495767913751, -196.0023115497991739 ) ) ;
#30992=CARTESIAN_POINT ( 'NONE',  ( 35.19605352522275155, -285.7294230312164700, -246.5069419418688028 ) ) ;
#30993=CARTESIAN_POINT ( 'NONE',  ( -6.905125520319645105, -284.2460515452305003, -337.6063407802757297 ) ) ;
#30994=CARTESIAN_POINT ( 'NONE',  ( 0.3460335736755167368, -280.7972168517744080, -336.3580293811020283 ) ) ;
#30995=CARTESIAN_POINT ( 'NONE',  ( -109.9728876694250630, -290.6488305719263394, -263.0323666336493034 ) ) ;
#30996=CARTESIAN_POINT ( 'NONE',  ( 7.487014525540851118, -282.1022584347446127, -211.9377555673985967 ) ) ;
#30997=CARTESIAN_POINT ( 'NONE',  ( -29.41702354663625485, -283.7521827771386143, -343.1427532545968120 ) ) ;
#30998=CARTESIAN_POINT ( 'NONE',  ( -56.84045206463820676, -291.2821259691905880, -343.2038134865892403 ) ) ;
#30999=CARTESIAN_POINT ( 'NONE',  ( -112.4236025583908827, -273.0978965691595022, -253.3772368265154284 ) ) ;
#31001=CARTESIAN_POINT ( 'NONE',  ( -73.75522819553066256, -287.6114785624052388, -336.5829098105638195 ) ) ;
#31002=CARTESIAN_POINT ( 'NONE',  ( 35.72995802030734325, -275.2446097838474088, -245.9127482146673742 ) ) ;
#31003=CARTESIAN_POINT ( 'NONE',  ( -89.08860771884337737, -293.3005492446556559, -216.4927803500606274 ) ) ;
#31005=CARTESIAN_POINT ( 'NONE',  ( 39.58706461736021254, -278.0519495502701943, -270.3284710469133074 ) ) ;
#31006=CARTESIAN_POINT ( 'NONE',  ( -112.5430771785299982, -276.5726598176918287, -268.7475629791378537 ) ) ;
#31008=CARTESIAN_POINT ( 'NONE',  ( -80.15848654505538207, -295.8832813941472182, -207.2646544771614003 ) ) ;
#31009=CARTESIAN_POINT ( 'NONE',  ( -93.85189590183601638, -272.5569400192231342, -223.9681668027124601 ) ) ;
#31010=CARTESIAN_POINT ( 'NONE',  ( -108.0661060631505421, -292.3441740029152811, -249.6096001975662659 ) ) ;
#31011=CARTESIAN_POINT ( 'NONE',  ( -107.2297361661133692, -291.7830566190655190, -248.4311625303689652 ) ) ;
#31012=CARTESIAN_POINT ( 'NONE',  ( -87.60073110271942198, -285.5250884443810833, -324.7635604935977653 ) ) ;
#31013=CARTESIAN_POINT ( 'NONE',  ( 30.36831092891625516, -294.5157216689004827, -234.8359552624269497 ) ) ;
#31014=CARTESIAN_POINT ( 'NONE',  ( 8.541702243843536380, -293.9807435108533582, -209.0740018201842076 ) ) ;
#31015=CARTESIAN_POINT ( 'NONE',  ( -35.65274239336272899, -294.8637293497181986, -343.3540733213288831 ) ) ;
#31016=CARTESIAN_POINT ( 'NONE',  ( 34.22966173808458734, -289.8434941295461158, -292.9515798301669065 ) ) ;
#31017=CARTESIAN_POINT ( 'NONE',  ( 37.67701682203558278, -281.5011298769188670, -252.9483071895343755 ) ) ;
#31018=CARTESIAN_POINT ( 'NONE',  ( -110.6174491953025552, -270.9391015437068972, -250.8999779970192492 ) ) ;
#31019=CARTESIAN_POINT ( 'NONE',  ( -63.19943619837910376, -285.5577499735842935, -197.8326581214946316 ) ) ;
#31020=CARTESIAN_POINT ( 'NONE',  ( 23.82788639542939535, -278.1164994543727289, -313.2298977835650362 ) ) ;
#31021=CARTESIAN_POINT ( 'NONE',  ( -89.93673888223572987, -284.0840889647931817, -219.0935482792116318 ) ) ;
#31022=CARTESIAN_POINT ( 'NONE',  ( 36.81209533043386983, -285.4066402843414494, -259.0408637420689502 ) ) ;
#31023=CARTESIAN_POINT ( 'NONE',  ( -25.56386379960523669, -278.3402871659473590, -195.5173603953421662 ) ) ;
#31025=CARTESIAN_POINT ( 'NONE',  ( -95.81142413951739911, -284.6742469950197005, -226.5515320925865694 ) ) ;
#31026=CARTESIAN_POINT ( 'NONE',  ( -17.11169846175850751, -281.5127730607071044, -196.4777250574909999 ) ) ;
#31027=CARTESIAN_POINT ( 'NONE',  ( 39.12144958106048875, -286.5184563743397916, -262.9918087221679457 ) ) ;
#31028=CARTESIAN_POINT ( 'NONE',  ( 21.34015577906363603, -295.9385735188422473, -315.4863527194883659 ) ) ;
#31029=CARTESIAN_POINT ( 'NONE',  ( -12.11164019505260114, -278.3294920447376057, -342.3183787250977730 ) ) ;
#31030=CARTESIAN_POINT ( 'NONE',  ( -90.97132770574519611, -279.1091573190154804, -324.9986601091004559 ) ) ;
#31031=CARTESIAN_POINT ( 'NONE',  ( -110.3919405749448828, -278.3818457035766301, -270.6359353346821877 ) ) ;
#31032=CARTESIAN_POINT ( 'NONE',  ( -37.17036250404844822, -300.0544674658183908, -195.5247971959151698 ) ) ;
#31033=CARTESIAN_POINT ( 'NONE',  ( 35.79301563801396924, -285.3479802380443857, -254.5073556351011348 ) ) ;
#31034=CARTESIAN_POINT ( 'NONE',  ( -113.3131159164553310, -292.0695748469799469, -276.9053817887482296 ) ) ;
#31035=CARTESIAN_POINT ( 'NONE',  ( -9.124555206144174591, -293.5946391394468833, -338.0358384481833696 ) ) ;
#31036=VERTEX_POINT ( 'NONE', #80778 ) ;
#31037=CARTESIAN_POINT ( 'NONE',  ( -35.65437969978824384, -294.6971551619258776, -343.3752645657835387 ) ) ;
#31039=CARTESIAN_POINT ( 'NONE',  ( -105.7346971997313432, -292.0816390355956855, -235.5468607831030567 ) ) ;
#31040=CARTESIAN_POINT ( 'NONE',  ( -46.47740995313754553, -280.5847093735756630, -197.7811118939073367 ) ) ;
#31041=CARTESIAN_POINT ( 'NONE',  ( -94.90208187056848033, -272.3007570314575219, -219.5711320898629424 ) ) ;
#31042=CARTESIAN_POINT ( 'NONE',  ( 39.25233834771363917, -288.1108650007719234, -262.9588120497893442 ) ) ;
#31043=CARTESIAN_POINT ( 'NONE',  ( -17.72561874659924186, -289.1391174892108893, -344.7987001751171761 ) ) ;
#31044=CARTESIAN_POINT ( 'NONE',  ( 18.67525144526882741, -287.2205446943539755, -223.4994722412025681 ) ) ;
#31046=CARTESIAN_POINT ( 'NONE',  ( 201.3567329005774127, 295.1815717130147050, -68.48326189999360736 ) ) ;
#31047=CARTESIAN_POINT ( 'NONE',  ( -89.29193934165813573, -229.1055583197461942, -344.3944809956333302 ) ) ;
#31048=CARTESIAN_POINT ( 'NONE',  ( -9.937345416836114609, -275.8820881573837482, -338.2098295645109260 ) ) ;
#31049=CARTESIAN_POINT ( 'NONE',  ( -66.94001918243773730, -276.3697760837334840, -337.4294829807162159 ) ) ;
#31050=CARTESIAN_POINT ( 'NONE',  ( -71.38962926465048042, -273.2814996947798818, -201.3213988842951494 ) ) ;
#31051=CARTESIAN_POINT ( 'NONE',  ( -54.13981448090132176, -170.3343158955618435, -361.5216119282826526 ) ) ;
#31053=CARTESIAN_POINT ( 'NONE',  ( -71.36667737921057153, -276.1769077074770280, -338.8855603213022505 ) ) ;
#31055=CARTESIAN_POINT ( 'NONE',  ( -78.20364462691486551, -290.1102090505617639, -330.9884301060386633 ) ) ;
#31056=CARTESIAN_POINT ( 'NONE',  ( -70.66827288754706160, -298.4265770473597286, -201.1260230554900943 ) ) ;
#31057=CARTESIAN_POINT ( 'NONE',  ( -78.79359665440387062, -274.1605715028558734, -205.5918887082693232 ) ) ;
#31058=CARTESIAN_POINT ( 'NONE',  ( -75.21245992568800887, -297.6991725676423357, -207.8941330934979703 ) ) ;
#31061=CARTESIAN_POINT ( 'NONE',  ( -95.03358613203458560, -279.8021199260835488, -319.1761667144942294 ) ) ;
#31062=CARTESIAN_POINT ( 'NONE',  ( -50.08949138887742691, -282.7181737146946148, -346.2899841551241025 ) ) ;
#31063=CARTESIAN_POINT ( 'NONE',  ( -94.68626719785807211, -278.9893310696669460, -316.0520169221155129 ) ) ;
#31064=CARTESIAN_POINT ( 'NONE',  ( -112.0649975234610451, -280.1365116622330333, -284.2311474986369717 ) ) ;
#31065=CARTESIAN_POINT ( 'NONE',  ( -111.0350334602965745, -271.0322748266905251, -270.3418080582339371 ) ) ;
#31068=CARTESIAN_POINT ( 'NONE',  ( -5.560412548954341005, -280.6489433850561568, -204.6424009808283984 ) ) ;
#31069=CARTESIAN_POINT ( 'NONE',  ( 38.02598496985002186, -276.5424985299037530, -285.3234327765041485 ) ) ;
#31070=CARTESIAN_POINT ( 'NONE',  ( 22.78008526482760487, -278.1646343248336279, -315.1982852973474678 ) ) ;
#31071=CARTESIAN_POINT ( 'NONE',  ( 38.79186051735894836, -274.2088363098354762, -276.8639815984653865 ) ) ;
#31074=CARTESIAN_POINT ( 'NONE',  ( -30.78233733491283530, -291.3343519672021671, -197.4942771925220484 ) ) ;
#31075=CARTESIAN_POINT ( 'NONE',  ( 22.91719306640145604, -286.2604194844438439, -222.5679743845104497 ) ) ;
#31076=CARTESIAN_POINT ( 'NONE',  ( -68.22738407053934395, -281.7033387046247412, -337.6221657255593414 ) ) ;
#31077=CARTESIAN_POINT ( 'NONE',  ( -65.55827921416104687, -282.0031993396327721, -338.3395216137096213 ) ) ;
#31078=CARTESIAN_POINT ( 'NONE',  ( 37.12148549603017500, -285.6052818854415136, -268.2964456424501805 ) ) ;
#31079=CARTESIAN_POINT ( 'NONE',  ( 6.088408726772941648, -290.4634891809606643, -331.5697826998103892 ) ) ;
#31080=CARTESIAN_POINT ( 'NONE',  ( 33.11145527166746660, -282.4864676467091726, -249.7824056915294477 ) ) ;
#31081=CARTESIAN_POINT ( 'NONE',  ( -95.37195680833850986, -271.2071589840551269, -222.8280344407132532 ) ) ;
#31082=CARTESIAN_POINT ( 'NONE',  ( -37.33499450532752206, -281.4519118874254673, -346.5740495856546204 ) ) ;
#31083=CARTESIAN_POINT ( 'NONE',  ( 14.12523251046627593, -296.3295367555321036, -324.9152699007491378 ) ) ;
#31084=CARTESIAN_POINT ( 'NONE',  ( -64.36077052982544444, -277.9443337727344101, -199.2849078251018966 ) ) ;
#31085=CARTESIAN_POINT ( 'NONE',  ( -78.68282330291975768, -278.2765235587290249, -330.7120894137035521 ) ) ;
#31086=CARTESIAN_POINT ( 'NONE',  ( -111.2017541711363577, -286.7345149946154947, -256.1355601458240585 ) ) ;
#31088=CARTESIAN_POINT ( 'NONE',  ( -36.42094875976950163, -293.9837602904037794, -194.7939360289124124 ) ) ;
#31089=CARTESIAN_POINT ( 'NONE',  ( -4.204748410161117000, -274.6152354737340033, -337.6579485607016409 ) ) ;
#31090=CARTESIAN_POINT ( 'NONE',  ( 19.49789741447913727, -287.4537028498629070, -322.0858286992382205 ) ) ;
#31091=CARTESIAN_POINT ( 'NONE',  ( 9.370793387368959060, -291.1060558259313780, -213.1600367166799685 ) ) ;
#31093=CARTESIAN_POINT ( 'NONE',  ( -59.35858162277882144, -276.0280705720673495, -340.4788789733017893 ) ) ;
#31094=CARTESIAN_POINT ( 'NONE',  ( -97.42180567627605114, -294.0914502449464294, -313.9861081809409598 ) ) ;
#31095=CARTESIAN_POINT ( 'NONE',  ( -109.9033482112654241, -291.7134588841587401, -282.1042400704192232 ) ) ;
#31098=CARTESIAN_POINT ( 'NONE',  ( 37.38689756574318324, -291.8363941073275214, -254.8585912475083717 ) ) ;
#31099=CARTESIAN_POINT ( 'NONE',  ( 36.48003702114210967, -289.1249978696617973, -268.2696779565584961 ) ) ;
#31100=CARTESIAN_POINT ( 'NONE',  ( -108.9186928366016360, -288.4639722891505471, -296.0262226212167320 ) ) ;
#31101=CARTESIAN_POINT ( 'NONE',  ( -10.55224504863196877, -287.8338716735656817, -201.8077148912684606 ) ) ;
#31103=CARTESIAN_POINT ( 'NONE',  ( 5.948384017670295343, -289.2511842730640410, -329.4036667606699211 ) ) ;
#31104=CARTESIAN_POINT ( 'NONE',  ( -47.38681910095937155, -297.1591099574680470, -345.0437959326230271 ) ) ;
#31106=CARTESIAN_POINT ( 'NONE',  ( -30.93244985530418489, -287.3364908038143426, -194.0135598770844467 ) ) ;
#31107=CARTESIAN_POINT ( 'NONE',  ( -71.73315828344635747, -277.6201419977205660, -203.2972893066325923 ) ) ;
#31108=CARTESIAN_POINT ( 'NONE',  ( -39.95798192828497974, -277.4174277667568731, -347.3085641051430343 ) ) ;
#31109=CARTESIAN_POINT ( 'NONE',  ( -4.949022481863993406, -280.1338350311138470, -200.5294723872359270 ) ) ;
#31110=CARTESIAN_POINT ( 'NONE',  ( -109.9446830035449096, -274.6849205963936242, -253.9257573333467803 ) ) ;
#31111=CARTESIAN_POINT ( 'NONE',  ( -7.434644306230026700, -284.4441421982089651, -201.5819884206332517 ) ) ;
#31113=CARTESIAN_POINT ( 'NONE',  ( 3.401376990437325887, -278.7454020324543649, -208.2440689300214558 ) ) ;
#31114=CARTESIAN_POINT ( 'NONE',  ( -41.48480965851955915, -281.1040366499012180, -345.2975657566988161 ) ) ;
#31116=CARTESIAN_POINT ( 'NONE',  ( -67.45299189145065100, -275.9199020261984856, -340.4754379337923069 ) ) ;
#31118=CARTESIAN_POINT ( 'NONE',  ( -92.69882106824934453, -297.3843667337218335, -319.0057159843598242 ) ) ;
#31119=CARTESIAN_POINT ( 'NONE',  ( -3.043468525732636820, -281.5300511094091007, -338.9696164472081250 ) ) ;
#31120=CARTESIAN_POINT ( 'NONE',  ( -98.92468540723368164, -296.9455227787425997, -310.0891370555709727 ) ) ;
#31121=CARTESIAN_POINT ( 'NONE',  ( -113.2791241367444428, -274.0844449043332247, -261.8691260446893239 ) ) ;
#31122=CARTESIAN_POINT ( 'NONE',  ( -92.03118050562272856, -272.9099756358900208, -221.9757046552343525 ) ) ;
#31123=CARTESIAN_POINT ( 'NONE',  ( -6.469640349231226217, -294.4577616547124990, -202.0096982667619159 ) ) ;
#31124=CARTESIAN_POINT ( 'NONE',  ( 39.35446176752952852, -287.6262099187212584, -262.9551506621767203 ) ) ;
#31126=CARTESIAN_POINT ( 'NONE',  ( -69.33007469440485693, -277.7144762720596987, -201.8922107046597603 ) ) ;
#31127=CARTESIAN_POINT ( 'NONE',  ( -94.70988830552268212, -291.0821642469255721, -219.0007150465193320 ) ) ;
#31128=CARTESIAN_POINT ( 'NONE',  ( -78.31595514275134917, -288.6768407134449035, -331.1224128368806419 ) ) ;
#31129=CARTESIAN_POINT ( 'NONE',  ( 36.87663642770926486, -291.4088359904366712, -259.2118925189142828 ) ) ;
#31132=CARTESIAN_POINT ( 'NONE',  ( -96.61220654691716447, -289.4628784095506830, -313.0810841650403518 ) ) ;
#31134=CARTESIAN_POINT ( 'NONE',  ( -29.49893008541301853, -287.0904414250848617, -193.9980957088475293 ) ) ;
#31135=CARTESIAN_POINT ( 'NONE',  ( -21.33282851196159058, -285.3376638359844719, -340.3538533559490702 ) ) ;
#31136=CARTESIAN_POINT ( 'NONE',  ( -53.25221955996107681, -294.3099916530228484, -345.5132698308053136 ) ) ;
#31137=CARTESIAN_POINT ( 'NONE',  ( 8.923979335357861586, -283.7473621979519294, -331.2937461487116479 ) ) ;
#31138=CARTESIAN_POINT ( 'NONE',  ( -82.79638025751717123, -283.5267814159249156, -327.5475390881124440 ) ) ;
#31139=CARTESIAN_POINT ( 'NONE',  ( -92.17055285695741418, -273.4614253745668293, -216.2982202343365827 ) ) ;
#31140=CARTESIAN_POINT ( 'NONE',  ( 23.45090834968755900, -276.2965725833308852, -229.0408253517988726 ) ) ;
#31141=CARTESIAN_POINT ( 'NONE',  ( -11.67140004799853514, -290.4080372402483476, -200.2140613158329643 ) ) ;
#31142=CARTESIAN_POINT ( 'NONE',  ( 3.161782837225202147, -273.4041933492162570, -209.0909061564801448 ) ) ;
#31143=ORIENTED_EDGE ( 'NONE', *, *, #13746, .T. ) ;
#31145=CARTESIAN_POINT ( 'NONE',  ( -68.16586294432359239, -287.5643137180773010, -202.6028329715966549 ) ) ;
#31146=CARTESIAN_POINT ( 'NONE',  ( -104.3261903770420815, -297.1444842018564145, -307.8135951936343986 ) ) ;
#31147=CARTESIAN_POINT ( 'NONE',  ( -108.4666152091295714, -285.4266680623216530, -253.4211180973144337 ) ) ;
#31149=CARTESIAN_POINT ( 'NONE',  ( -99.46642073409125828, -277.0105674942417409, -315.4760379398939563 ) ) ;
#31150=CARTESIAN_POINT ( 'NONE',  ( 36.18708073237117162, -293.9205021860741454, -247.8482067582093293 ) ) ;
#31151=CARTESIAN_POINT ( 'NONE',  ( 11.30295960121781640, -284.8571288396806267, -212.2064757025541439 ) ) ;
#31152=CARTESIAN_POINT ( 'NONE',  ( -4.507698627687532600, -294.9645524544523028, -340.0008142084745373 ) ) ;
#31153=CARTESIAN_POINT ( 'NONE',  ( -52.37826750909458440, -292.1876674294911709, -198.8529971689560512 ) ) ;
#31156=CARTESIAN_POINT ( 'NONE',  ( -11.83151317026870863, -92.77902702734904494, -356.4673753602164084 ) ) ;
#31157=CARTESIAN_POINT ( 'NONE',  ( -113.1332553958814060, -286.1839767811628121, -261.5096829539981513 ) ) ;
#31158=CARTESIAN_POINT ( 'NONE',  ( -85.33152481854864391, -293.1952119285920162, -330.4860931364850671 ) ) ;
#31160=CARTESIAN_POINT ( 'NONE',  ( -67.92580901613808919, -282.3836984344101211, -336.9857257343207948 ) ) ;
#31161=CARTESIAN_POINT ( 'NONE',  ( -111.8080682624107709, -277.9740491756704728, -289.9194430079709832 ) ) ;
#31162=CARTESIAN_POINT ( 'NONE',  ( 33.70943723173035522, -283.2462194378555864, -246.7083055832999605 ) ) ;
#31163=CARTESIAN_POINT ( 'NONE',  ( 203.5065358818463039, 290.8197351118913616, -82.79791085622774460 ) ) ;
#31164=CARTESIAN_POINT ( 'NONE',  ( -10.92292360015097863, -281.2892216431121142, -342.1156832415301778 ) ) ;
#31165=CARTESIAN_POINT ( 'NONE',  ( 35.60872053726603070, -285.3682452542266788, -254.5471073751929225 ) ) ;
#31166=CARTESIAN_POINT ( 'NONE',  ( -32.78101520179771455, -275.9694312606602011, -194.7207649540964951 ) ) ;
#31167=CARTESIAN_POINT ( 'NONE',  ( -110.4359676837275117, -297.0658990923544138, -268.7377798556076414 ) ) ;
#31168=CARTESIAN_POINT ( 'NONE',  ( 34.97139959636359663, -292.0641807090532325, -257.1739236609606678 ) ) ;
#31169=CARTESIAN_POINT ( 'NONE',  ( -77.75426505457394910, -278.2307938404647984, -335.8457519960007858 ) ) ;
#31170=CARTESIAN_POINT ( 'NONE',  ( -59.19499859944602349, -277.3430327698906126, -340.0133494322519141 ) ) ;
#31171=CARTESIAN_POINT ( 'NONE',  ( -89.96081201947748696, -274.4097504971363151, -214.4968149782511375 ) ) ;
#31172=CARTESIAN_POINT ( 'NONE',  ( -89.01402651425053136, -276.6789528308228796, -327.0308911854293115 ) ) ;
#31173=CARTESIAN_POINT ( 'NONE',  ( 138.5464852710080379, 180.7133914993734436, -241.3450704664923023 ) ) ;
#31174=CARTESIAN_POINT ( 'NONE',  ( 25.34202474789456616, -274.1087936162026040, -311.6327664301645655 ) ) ;
#31176=CARTESIAN_POINT ( 'NONE',  ( -30.62453176540203614, -296.3940587629892889, -346.4760701393184377 ) ) ;
#31179=CARTESIAN_POINT ( 'NONE',  ( -93.65071082920812273, -284.9685253581998836, -317.3027986978677291 ) ) ;
#31180=CARTESIAN_POINT ( 'NONE',  ( -109.2583027693600428, -285.9990202902943111, -294.8963228410667625 ) ) ;
#31181=CARTESIAN_POINT ( 'NONE',  ( -60.00236293355126804, -285.0991491072461486, -200.8601321678202112 ) ) ;
#31182=CARTESIAN_POINT ( 'NONE',  ( -109.5517186309650697, -276.7532046744018999, -285.5977070091549308 ) ) ;
#31183=CARTESIAN_POINT ( 'NONE',  ( -111.0971906121151136, -286.2975372072384062, -279.2290373385666271 ) ) ;
#31184=CARTESIAN_POINT ( 'NONE',  ( -85.92690563530614156, -277.8442349794473785, -214.9518628300086220 ) ) ;
#31185=CARTESIAN_POINT ( 'NONE',  ( -18.92607358121420091, -277.8891153793734361, -341.3194914952528052 ) ) ;
#31187=CARTESIAN_POINT ( 'NONE',  ( -35.39496626076196151, -274.5695560508064546, -197.3130034089043363 ) ) ;
#31189=CARTESIAN_POINT ( 'NONE',  ( 8.442107870269278891, -281.4637397830929331, -208.5859754575935199 ) ) ;
#31190=CARTESIAN_POINT ( 'NONE',  ( -28.23851193312138363, -280.6569362847545790, -193.9095071544167865 ) ) ;
#31194=CARTESIAN_POINT ( 'NONE',  ( 35.20954916508422627, -289.6915559102340580, -292.2378930924705287 ) ) ;
#31195=CARTESIAN_POINT ( 'NONE',  ( -98.57713424454352946, -296.3040376577786219, -230.2341828547328646 ) ) ;
#31196=CARTESIAN_POINT ( 'NONE',  ( -88.57538942831727979, -290.7040064570267646, -213.0163547779379769 ) ) ;
#31197=CARTESIAN_POINT ( 'NONE',  ( 35.96606130279737812, -285.9336434222134358, -262.8325148160609501 ) ) ;
#31198=CARTESIAN_POINT ( 'NONE',  ( -3.108310395638296697, -287.1656985107426863, -335.5593133010006568 ) ) ;
#31199=CARTESIAN_POINT ( 'NONE',  ( -49.50234660859983649, -287.0988731822736213, -197.9266796547319132 ) ) ;
#31200=CARTESIAN_POINT ( 'NONE',  ( -69.46805234446085819, -275.4747023220432993, -338.1461062446286974 ) ) ;
#31201=CARTESIAN_POINT ( 'NONE',  ( 29.64955561954562313, -286.4279818388127410, -306.7841156911260896 ) ) ;
#31202=CARTESIAN_POINT ( 'NONE',  ( 8.565927474749594595, -288.6812277543717187, -211.0526837296688996 ) ) ;
#31203=CARTESIAN_POINT ( 'NONE',  ( -77.18670593061705176, -287.5843468117639645, -334.1588359666959605 ) ) ;
#31204=CARTESIAN_POINT ( 'NONE',  ( -45.65430985022116062, -284.1012085413401564, -343.1742780628101741 ) ) ;
#31205=CARTESIAN_POINT ( 'NONE',  ( -112.2824234709824083, -292.4695425225361305, -276.8219813907830940 ) ) ;
#31208=CARTESIAN_POINT ( 'NONE',  ( -37.27978344253750009, -299.9730717146126153, -194.8003405251599816 ) ) ;
#31209=CARTESIAN_POINT ( 'NONE',  ( 33.27211649700328167, -280.4964862288603058, -251.1744415036023952 ) ) ;
#31210=CARTESIAN_POINT ( 'NONE',  ( 35.71418299237766547, -279.3341532064007993, -253.3953113404013777 ) ) ;
#31211=CARTESIAN_POINT ( 'NONE',  ( 23.03842418190843588, -293.3864071452224493, -317.9048447339581003 ) ) ;
#31212=CARTESIAN_POINT ( 'NONE',  ( -85.95915093221232439, -271.6078548603810532, -214.4867573899274760 ) ) ;
#31213=CARTESIAN_POINT ( 'NONE',  ( 37.13922741289556484, -273.6484516620014915, -271.6335103043355161 ) ) ;
#31214=CARTESIAN_POINT ( 'NONE',  ( -105.4124117120327071, -297.4986762830105818, -298.0671047246954686 ) ) ;
#31216=CARTESIAN_POINT ( 'NONE',  ( -85.42327959076786215, -271.9769064233275344, -210.9745201034476736 ) ) ;
#31217=CARTESIAN_POINT ( 'NONE',  ( -104.3493041490805808, -295.2625406826643939, -234.4172416969004189 ) ) ;
#31218=CARTESIAN_POINT ( 'NONE',  ( 23.82096670782933856, -294.4136692671864921, -229.4404251394196592 ) ) ;
#31219=CARTESIAN_POINT ( 'NONE',  ( 104.2209783822911646, -299.5541904835127980, -193.4627128438320938 ) ) ;
#31220=CARTESIAN_POINT ( 'NONE',  ( 27.30553509052749916, -294.8218637758599243, -304.7234052940085007 ) ) ;
#31221=PLANE ( 'NONE',  #71676 ) ;
#31222=CARTESIAN_POINT ( 'NONE',  ( -49.06345900759774281, -283.9237579926843296, -195.8705901125350124 ) ) ;
#31223=CARTESIAN_POINT ( 'NONE',  ( 28.39455219974218636, -293.9831561068069163, -302.2226944999908937 ) ) ;
#31224=CARTESIAN_POINT ( 'NONE',  ( -24.53358155959462295, -282.8931503969599817, -346.3425155850067654 ) ) ;
#31225=CARTESIAN_POINT ( 'NONE',  ( 20.84585023827576578, -282.8119220947845065, -222.1581804790805279 ) ) ;
#31226=CARTESIAN_POINT ( 'NONE',  ( -99.32468945516025371, -284.8265113520943714, -224.6241757582789376 ) ) ;
#31227=CARTESIAN_POINT ( 'NONE',  ( -89.18272769446753045, -289.3211376649276190, -216.3216111355461635 ) ) ;
#31228=CARTESIAN_POINT ( 'NONE',  ( 36.51581113150614044, -280.2742441802406006, -289.5385991784507382 ) ) ;
#31229=CARTESIAN_POINT ( 'NONE',  ( -8.043061220241614961, -285.1290179622242817, -202.9605746822465449 ) ) ;
#31230=CARTESIAN_POINT ( 'NONE',  ( -5.766373805197273938, -287.5669366634023163, -340.2502536075998592 ) ) ;
#31232=CARTESIAN_POINT ( 'NONE',  ( -90.97476348873112784, -297.4292653437055378, -321.1292158681425235 ) ) ;
#31233=CARTESIAN_POINT ( 'NONE',  ( -99.97205941160669340, -279.3942942482120202, -314.1337622856285066 ) ) ;
#31234=CARTESIAN_POINT ( 'NONE',  ( -44.66149869112747695, -293.1643213388960021, -345.4122336924806405 ) ) ;
#31235=CARTESIAN_POINT ( 'NONE',  ( -37.00397014956839570, -279.7232146820932712, -197.3407548956787707 ) ) ;
#31236=CARTESIAN_POINT ( 'NONE',  ( -40.63454460683927039, -292.1785230287092077, -193.4183759349064644 ) ) ;
#31237=CARTESIAN_POINT ( 'NONE',  ( -92.84503817647167523, -283.3441119471802949, -219.0136775605955393 ) ) ;
#31238=CARTESIAN_POINT ( 'NONE',  ( -53.67034497485278166, -279.2617067203428292, -343.6152644030746046 ) ) ;
#31239=CARTESIAN_POINT ( 'NONE',  ( -26.18334357592893724, -293.9653473019334342, -342.7413606365951750 ) ) ;
#31240=CARTESIAN_POINT ( 'NONE',  ( -96.35744694540538546, -271.1898637039643631, -223.8082441841174841 ) ) ;
#31243=CARTESIAN_POINT ( 'NONE',  ( 35.84830915361725800, -283.7220711181074080, -285.0907916521785523 ) ) ;
#31244=CARTESIAN_POINT ( 'NONE',  ( -96.46189878924629113, -295.4592979281346743, -313.3102106603600987 ) ) ;
#31246=CARTESIAN_POINT ( 'NONE',  ( 35.78497577281001440, -272.8380690714490129, -253.7030783399848985 ) ) ;
#31247=CARTESIAN_POINT ( 'NONE',  ( 9.420182046173946944, -273.8739431225682210, -209.3899346618975983 ) ) ;
#31248=CARTESIAN_POINT ( 'NONE',  ( -17.83380835474038051, -290.1208522788536470, -344.3390905827596953 ) ) ;
#31249=CARTESIAN_POINT ( 'NONE',  ( -97.35011842549882033, -289.8060457459617396, -311.9521759493230775 ) ) ;
#31250=CARTESIAN_POINT ( 'NONE',  ( -68.83701028284195900, -281.1504719300153283, -203.7371493759753491 ) ) ;
#31251=CARTESIAN_POINT ( 'NONE',  ( -34.45244230781214867, -299.8489447999542108, -196.3468973494859995 ) ) ;
#31252=CARTESIAN_POINT ( 'NONE',  ( 0.6183820539838543739, -279.3649575833840117, -207.4837887910809116 ) ) ;
#31254=CARTESIAN_POINT ( 'NONE',  ( 7.236718122286518451, -274.4741414487317002, -207.5122079605968679 ) ) ;
#31255=CARTESIAN_POINT ( 'NONE',  ( -68.42432604560799803, -293.5607539032566820, -202.7069995643404354 ) ) ;
#31257=CARTESIAN_POINT ( 'NONE',  ( -107.8218623798989739, -290.9453473960938368, -289.9496252828471938 ) ) ;
#31260=CARTESIAN_POINT ( 'NONE',  ( -41.95470197703103565, -290.1341792296234416, -194.7368778520182104 ) ) ;
#31261=CARTESIAN_POINT ( 'NONE',  ( -47.27142345842409554, -297.5893604061282076, -197.9670419624538908 ) ) ;
#31263=CARTESIAN_POINT ( 'NONE',  ( -104.0136727477975427, -292.5577853298449895, -233.2456789020233714 ) ) ;
#31264=CARTESIAN_POINT ( 'NONE',  ( 36.57525178469696669, -295.6233781216987495, -234.7283546768995564 ) ) ;
#31265=CARTESIAN_POINT ( 'NONE',  ( 8.018469824741391250, -288.6734769092363990, -210.7768981873759628 ) ) ;
#31266=CARTESIAN_POINT ( 'NONE',  ( 17.86692047987866516, -274.2591556020927328, -320.8979091396874423 ) ) ;
#31267=CARTESIAN_POINT ( 'NONE',  ( 32.46028268355424728, -277.1340675933158195, -244.4961340879069951 ) ) ;
#31268=CARTESIAN_POINT ( 'NONE',  ( -14.37942983481254977, -290.4320455851233191, -199.5511727832560496 ) ) ;
#31269=CARTESIAN_POINT ( 'NONE',  ( -58.97252696514448900, -281.6356091029114737, -197.7497358952096533 ) ) ;
#31271=CARTESIAN_POINT ( 'NONE',  ( -16.11080883092867566, -282.1188305920303492, -340.3121145634739264 ) ) ;
#31272=CARTESIAN_POINT ( 'NONE',  ( -56.83214239136744084, -278.3773058576832113, -344.5888202230518687 ) ) ;
#31273=CARTESIAN_POINT ( 'NONE',  ( 27.95844798005542486, -280.8742149126379672, -310.5103224392374273 ) ) ;
#31274=CARTESIAN_POINT ( 'NONE',  ( -99.45230775254184152, -278.8927673148161261, -315.4954661341138831 ) ) ;
#31278=CARTESIAN_POINT ( 'NONE',  ( -10.60881529658629496, -275.9146046465056656, -198.8342137008324073 ) ) ;
#31279=CARTESIAN_POINT ( 'NONE',  ( -21.39648532958013050, -282.7662352645559167, -200.3538533559491555 ) ) ;
#31281=CARTESIAN_POINT ( 'NONE',  ( -101.6237757677808986, -299.0709051315496936, -231.6230966172172430 ) ) ;
#31282=CARTESIAN_POINT ( 'NONE',  ( -80.57877697352100199, -290.7333530767123193, -329.6254709182156262 ) ) ;
#31283=CARTESIAN_POINT ( 'NONE',  ( -9.395449196819786408, -274.7052185775245903, -339.5909813700837390 ) ) ;
#31284=CARTESIAN_POINT ( 'NONE',  ( -68.91552868352297878, -291.2217299888569642, -339.4916815754901336 ) ) ;
#31285=CARTESIAN_POINT ( 'NONE',  ( -83.88756866074173502, -290.7414634574321894, -213.9929107166604467 ) ) ;
#31286=CARTESIAN_POINT ( 'NONE',  ( 7.893261822244963533, -287.9604855583655194, -332.6628565060133838 ) ) ;
#31288=CARTESIAN_POINT ( 'NONE',  ( -111.0256223141635701, -283.0168666224920457, -265.3912475153069863 ) ) ;
#31289=CARTESIAN_POINT ( 'NONE',  ( -101.3573071612549228, -291.9038145931454551, -308.0504411687865627 ) ) ;
#31290=CARTESIAN_POINT ( 'NONE',  ( -72.68973029123750962, -284.0549842843161628, -205.6843793963161886 ) ) ;
#31291=CARTESIAN_POINT ( 'NONE',  ( 34.81525019566386447, -282.6836656551529359, -256.3443409853006187 ) ) ;
#31292=CARTESIAN_POINT ( 'NONE',  ( 10.09199640086744587, -289.3579276242612082, -330.7848990320379130 ) ) ;
#31293=CARTESIAN_POINT ( 'NONE',  ( -99.52339878206137769, -279.5741387030121246, -231.9054346753736411 ) ) ;
#31294=CARTESIAN_POINT ( 'NONE',  ( 20.09121300513437447, -291.6569570679810681, -219.6513636628694428 ) ) ;
#31295=CARTESIAN_POINT ( 'NONE',  ( 37.55992325945679511, -288.1394652339694744, -253.1590818707464337 ) ) ;
#31296=CARTESIAN_POINT ( 'NONE',  ( -80.90852564738108299, -285.9706911173383332, -206.8818360392764930 ) ) ;
#31297=CARTESIAN_POINT ( 'NONE',  ( -109.1934052502100343, -284.8898934772623761, -257.3937898013255108 ) ) ;
#31300=CARTESIAN_POINT ( 'NONE',  ( 22.97723650387827732, -294.7913752883952725, -224.4929519617171252 ) ) ;
#31301=CARTESIAN_POINT ( 'NONE',  ( 22.77371527930553796, -292.8741486487296584, -317.7048016249416378 ) ) ;
#31302=CARTESIAN_POINT ( 'NONE',  ( 13.88738263509119086, -275.3710236332801173, -322.7670890616820998 ) ) ;
#31303=CARTESIAN_POINT ( 'NONE',  ( -112.1732452021648641, -296.1225054174698812, -252.6537000746140791 ) ) ;
#31304=CARTESIAN_POINT ( 'NONE',  ( 14.79322916045861369, -292.7814551397851801, -322.5160201341722654 ) ) ;
#31305=CARTESIAN_POINT ( 'NONE',  ( -103.6863120016833051, -294.3520135529505524, -303.2850293362074012 ) ) ;
#31306=CARTESIAN_POINT ( 'NONE',  ( -25.35930366297356287, -293.4132292720378814, -197.8969816658561456 ) ) ;
#31307=CARTESIAN_POINT ( 'NONE',  ( 31.83630369331150334, -294.9550604965350544, -294.7748942167126529 ) ) ;
#31309=CARTESIAN_POINT ( 'NONE',  ( -17.02742956347599801, -292.7904386131637011, -342.7846286132735827 ) ) ;
#31311=CARTESIAN_POINT ( 'NONE',  ( 16.19112397825171712, -289.2105433594653050, -320.4117799789893297 ) ) ;
#31312=CARTESIAN_POINT ( 'NONE',  ( -50.98944473884495210, -279.2056272548633160, -344.4701313819831512 ) ) ;
#31313=CARTESIAN_POINT ( 'NONE',  ( -100.1487843025347644, -276.7643709037999429, -314.2163217372786335 ) ) ;
#31314=CARTESIAN_POINT ( 'NONE',  ( -24.16889770465336440, -273.5645834375325194, -194.5456202010801405 ) ) ;
#31315=CARTESIAN_POINT ( 'NONE',  ( 30.61933368207897033, -280.0346027905635538, -300.8621172427498323 ) ) ;
#31316=CARTESIAN_POINT ( 'NONE',  ( -99.82135192412037838, -276.3693820378550754, -313.9814518576292812 ) ) ;
#31317=CARTESIAN_POINT ( 'NONE',  ( -108.7823309496259583, -295.0102832051042014, -287.6618377572248733 ) ) ;
#31318=CARTESIAN_POINT ( 'NONE',  ( -109.9191433715138260, -274.7976242761124013, -251.2551911447443160 ) ) ;
#31319=CARTESIAN_POINT ( 'NONE',  ( -97.93232411612436294, -273.7723056108166588, -229.3725214794351359 ) ) ;
#31321=CARTESIAN_POINT ( 'NONE',  ( -98.54933269549042052, -287.9767292865842023, -314.3381270416014104 ) ) ;
#31322=CARTESIAN_POINT ( 'NONE',  ( -16.63863031486884125, -274.1603750621654854, -200.3056741016278011 ) ) ;
#31323=CARTESIAN_POINT ( 'NONE',  ( 24.14220891692059467, -288.1694072093703767, -316.7155021176763512 ) ) ;
#31324=CARTESIAN_POINT ( 'NONE',  ( -43.18785736984990109, -299.9587091203084697, -195.1809583684856761 ) ) ;
#31325=CARTESIAN_POINT ( 'NONE',  ( -91.75744731388762432, -293.8295572231668871, -321.8065322391738619 ) ) ;
#31326=CARTESIAN_POINT ( 'NONE',  ( -18.96693985425484641, -282.0187456948979161, -345.0251203911348057 ) ) ;
#31327=CARTESIAN_POINT ( 'NONE',  ( 133.0872704186301405, -299.5541904835127980, -201.0153591320744226 ) ) ;
#31328=CARTESIAN_POINT ( 'NONE',  ( 36.55979728763310987, -279.3868304103137348, -257.4979387412158758 ) ) ;
#31330=CARTESIAN_POINT ( 'NONE',  ( -110.0915946498853941, -289.4796095885238287, -260.2593394080383860 ) ) ;
#31331=CARTESIAN_POINT ( 'NONE',  ( -111.5546622729918340, -282.6488063448979915, -273.6699567034181655 ) ) ;
#31333=LINE ( 'NONE', #44590, #62460 ) ;
#31334=CARTESIAN_POINT ( 'NONE',  ( -112.3065576144171303, -288.5055117251473575, -273.9807582936405197 ) ) ;
#31335=CARTESIAN_POINT ( 'NONE',  ( 21.22083368778951140, -276.4488238660761112, -225.6062794130096734 ) ) ;
#31336=CARTESIAN_POINT ( 'NONE',  ( -41.53198949850408894, -284.3087552535243390, -346.9014108187861893 ) ) ;
#31337=CARTESIAN_POINT ( 'NONE',  ( -24.38207594446435067, -272.2960468025480623, -195.8676344309231752 ) ) ;
#31338=CARTESIAN_POINT ( 'NONE',  ( -108.0286609912364781, -284.7928116850294487, -252.1305512351773075 ) ) ;
#31339=CARTESIAN_POINT ( 'NONE',  ( 27.29290080409853303, -277.4550709852956061, -305.6492667356996549 ) ) ;
#31340=CARTESIAN_POINT ( 'NONE',  ( -59.23359976853490849, -278.1457360501477751, -340.1704759280403891 ) ) ;
#31342=CARTESIAN_POINT ( 'NONE',  ( 3.479076350669284778, -284.5038572347049239, -333.3404328310936648 ) ) ;
#31345=CARTESIAN_POINT ( 'NONE',  ( -84.18688560425368905, -295.5093345531158207, -331.5391345022632663 ) ) ;
#31346=CARTESIAN_POINT ( 'NONE',  ( -5.110769517629338843, -288.4583207594378109, -203.0193643251922992 ) ) ;
#31348=CARTESIAN_POINT ( 'NONE',  ( -19.11405058567864046, -286.3380690714489560, -350.3683826091709648 ) ) ;
#31349=CARTESIAN_POINT ( 'NONE',  ( -113.4611929476531174, -277.3498624389717975, -280.1264454285906140 ) ) ;
#31350=CARTESIAN_POINT ( 'NONE',  ( -105.2815048512349563, -289.4022704879004095, -235.7394253883467456 ) ) ;
#31351=CARTESIAN_POINT ( 'NONE',  ( -57.60342536166332650, -287.3060447177883248, -199.4548406257005411 ) ) ;
#31352=CARTESIAN_POINT ( 'NONE',  ( -98.84803361238770947, -280.8773303680115419, -229.1003657316499869 ) ) ;
#31353=CARTESIAN_POINT ( 'NONE',  ( -37.99575236323442340, -287.4693738490169608, -193.9531438499307683 ) ) ;
#31354=CARTESIAN_POINT ( 'NONE',  ( -36.13653011754616529, -285.0371959870591922, -345.3514388110838809 ) ) ;
#31355=CARTESIAN_POINT ( 'NONE',  ( 38.18278396775849615, -275.9064488567860849, -285.3628614340199192 ) ) ;
#31356=CARTESIAN_POINT ( 'NONE',  ( 98.17144688861017698, -297.7765669504339598, -195.7623448073262864 ) ) ;
#31357=CARTESIAN_POINT ( 'NONE',  ( -111.7304775296174739, -278.6349930195842148, -250.4278200547514075 ) ) ;
#31358=CARTESIAN_POINT ( 'NONE',  ( -111.1675577024199839, -298.6008049307869783, -260.4283685838656766 ) ) ;
#31360=CARTESIAN_POINT ( 'NONE',  ( 10.64812456238590066, -278.9090924074130839, -330.4860931364851808 ) ) ;
#31361=CARTESIAN_POINT ( 'NONE',  ( -111.4499704650455811, -271.0048131427265616, -253.5700999803765967 ) ) ;
#31363=CARTESIAN_POINT ( 'NONE',  ( -66.83324651431099994, -276.9570053283635502, -337.2059916346631212 ) ) ;
#31364=CARTESIAN_POINT ( 'NONE',  ( 21.53577255653188161, -276.0946615466802427, -221.3565066662580705 ) ) ;
#31365=CARTESIAN_POINT ( 'NONE',  ( 38.56391707517012435, -280.4629069489377002, -258.5636069471576093 ) ) ;
#31366=CARTESIAN_POINT ( 'NONE',  ( 30.36094334646875481, -289.7107298007793474, -300.3936460072927161 ) ) ;
#31367=CARTESIAN_POINT ( 'NONE',  ( -113.6448539439465151, -298.0815165947082050, -269.6286777872169864 ) ) ;
#31368=CARTESIAN_POINT ( 'NONE',  ( -110.8300958887223260, -297.4840826714466289, -292.0282776306052597 ) ) ;
#31369=CARTESIAN_POINT ( 'NONE',  ( 35.42463123688356319, -295.3268785481492387, -252.8396441722057659 ) ) ;
#31370=CARTESIAN_POINT ( 'NONE',  ( 37.35128208426909424, -279.4930349272282797, -265.7799792356038893 ) ) ;
#31371=CARTESIAN_POINT ( 'NONE',  ( -34.27806860675843126, -282.0110912056253483, -195.9713925258860172 ) ) ;
#31372=CARTESIAN_POINT ( 'NONE',  ( -33.69993651244328703, -296.1779303398994898, -195.9223127172270438 ) ) ;
#31373=CARTESIAN_POINT ( 'NONE',  ( -103.3576731478390798, -286.6533841931981783, -232.1991869681958747 ) ) ;
#31374=CARTESIAN_POINT ( 'NONE',  ( -37.28150989865982723, -287.9717079146420815, -343.6702064497233664 ) ) ;
#31375=CARTESIAN_POINT ( 'NONE',  ( -62.00093947437260056, -183.6896612128238928, -362.0872038736079617 ) ) ;
#31377=CARTESIAN_POINT ( 'NONE',  ( 21.02709260368700939, -286.7963858990431731, -319.6732902074080584 ) ) ;
#31378=CARTESIAN_POINT ( 'NONE',  ( -9.481395755719859153, -286.0932452481566202, -202.8502656237699853 ) ) ;
#31380=CARTESIAN_POINT ( 'NONE',  ( -93.19694380638489406, -284.9114449797202155, -322.9320957600143629 ) ) ;
#31381=CARTESIAN_POINT ( 'NONE',  ( -8.966531441369978594, -274.7669419603913639, -203.0246740735224193 ) ) ;
#31382=CARTESIAN_POINT ( 'NONE',  ( -98.94804093791375976, -290.0823899216254063, -224.6647188990842210 ) ) ;
#31383=CARTESIAN_POINT ( 'NONE',  ( -5.490159567272129948, -283.2954408411344502, -340.3524899572649929 ) ) ;
#31384=CARTESIAN_POINT ( 'NONE',  ( -7.823235954678832371, -281.9520960981986377, -199.9809875617134196 ) ) ;
#31385=CARTESIAN_POINT ( 'NONE',  ( 8.530534332706116274, -280.9942639501025496, -208.4767199512577918 ) ) ;
#31386=CARTESIAN_POINT ( 'NONE',  ( -49.14190916843124057, -279.8975725031252750, -198.3211633281875095 ) ) ;
#31387=CARTESIAN_POINT ( 'NONE',  ( -69.91165696735023971, -274.9809262143061233, -337.9199732462171255 ) ) ;
#31388=CARTESIAN_POINT ( 'NONE',  ( -63.20851169538713066, -183.0927275039082929, -362.5798909104344148 ) ) ;
#31390=CARTESIAN_POINT ( 'NONE',  ( 29.48737834821474380, -277.1064677590645147, -236.6876463258043657 ) ) ;
#31391=CARTESIAN_POINT ( 'NONE',  ( 160.2970747563815053, 220.5528797148367914, -204.9019708605778192 ) ) ;
#31392=CARTESIAN_POINT ( 'NONE',  ( 22.30946005225842654, -280.1887542401478868, -315.2552285546606754 ) ) ;
#31393=CARTESIAN_POINT ( 'NONE',  ( -40.51410305601200434, -297.3598283656597800, -197.3154870207346505 ) ) ;
#31394=CARTESIAN_POINT ( 'NONE',  ( 11.08492328142546057, -292.2094548641217671, -210.5063748351800257 ) ) ;
#31395=CARTESIAN_POINT ( 'NONE',  ( 174.1105135456895141, 240.3386868887248511, -177.2113801460971558 ) ) ;
#31396=CARTESIAN_POINT ( 'NONE',  ( 75.32416697583983023, -298.0113065177353064, -193.9769740307470727 ) ) ;
#31397=CARTESIAN_POINT ( 'NONE',  ( -18.28637951969112407, -287.2024918181344901, -341.7117878292757496 ) ) ;
#31398=CARTESIAN_POINT ( 'NONE',  ( -105.0537192503782080, -298.0080034793483605, -300.9160769104076394 ) ) ;
#31399=CARTESIAN_POINT ( 'NONE',  ( -11.86663911566776441, -287.7060512650919009, -201.4244459977876716 ) ) ;
#31401=CARTESIAN_POINT ( 'NONE',  ( 36.47459659255399345, -294.2279168117560744, -249.2425444003685868 ) ) ;
#31402=CARTESIAN_POINT ( 'NONE',  ( -105.6246715811924872, -285.3912006289635883, -244.3721924357102750 ) ) ;
#31403=CARTESIAN_POINT ( 'NONE',  ( -36.88430695734270159, -296.8526895307199993, -193.7582787832450606 ) ) ;
#31404=CARTESIAN_POINT ( 'NONE',  ( -5.962255238215237618, -293.2570323792476188, -200.2077897503053521 ) ) ;
#31406=CARTESIAN_POINT ( 'NONE',  ( 36.64325970093131701, -293.7790845188023354, -249.2002724160592209 ) ) ;
#31407=CARTESIAN_POINT ( 'NONE',  ( -48.05888581371884527, -289.3588382067932798, -342.6211554911231474 ) ) ;
#31408=VERTEX_POINT ( 'NONE', #11015 ) ;
#31410=CARTESIAN_POINT ( 'NONE',  ( -4.110268410051605592, -300.3243722564834002, -194.5859091532147147 ) ) ;
#31411=CARTESIAN_POINT ( 'NONE',  ( -55.22595221914062336, -272.6219663342944273, -195.8751310816175817 ) ) ;
#31413=CARTESIAN_POINT ( 'NONE',  ( 7.930036280584154440, -281.4751049847474178, -327.9921712432815184 ) ) ;
#31416=CARTESIAN_POINT ( 'NONE',  ( -62.39188600105975269, -276.8770022920694487, -343.1636206328474259 ) ) ;
#31417=CARTESIAN_POINT ( 'NONE',  ( -109.3105731355164210, -271.1652082560592589, -254.0233783641224647 ) ) ;
#31418=CARTESIAN_POINT ( 'NONE',  ( -110.3511368125342074, -280.5868456490927088, -256.9265492439108698 ) ) ;
#31419=CARTESIAN_POINT ( 'NONE',  ( -0.8839295421733401881, -274.7026093141018919, -335.0853164081544264 ) ) ;
#31420=CARTESIAN_POINT ( 'NONE',  ( -86.37690161627159569, -298.5581431460211093, -215.7472047472665793 ) ) ;
#31421=CARTESIAN_POINT ( 'NONE',  ( -92.20234635300101900, -274.1843029003908896, -221.8459868964510235 ) ) ;
#31422=CARTESIAN_POINT ( 'NONE',  ( -112.4121267558787594, -297.9833166610093258, -283.7306166818533484 ) ) ;
#31423=CARTESIAN_POINT ( 'NONE',  ( -62.97341230813007229, -271.7401380474320831, -199.4991244121179648 ) ) ;
#31424=CARTESIAN_POINT ( 'NONE',  ( 35.39587545370003596, -294.1011036362260711, -262.5828358792764448 ) ) ;
#31425=CARTESIAN_POINT ( 'NONE',  ( 11.33404425929101045, -291.3168758948906429, -215.1021025869179653 ) ) ;
#31427=CARTESIAN_POINT ( 'NONE',  ( 31.80273434438988289, -276.4794517932647864, -304.2252508412464067 ) ) ;
#31428=CARTESIAN_POINT ( 'NONE',  ( -59.47766265483444670, -273.9242104854262720, -200.7452806851144089 ) ) ;
#31429=CARTESIAN_POINT ( 'NONE',  ( -68.99779512676353477, -282.1446124273924738, -340.0259254832058105 ) ) ;
#31430=CARTESIAN_POINT ( 'NONE',  ( 5.588328626319332137, -296.4728186242994639, -332.1257779332538576 ) ) ;
#31432=CARTESIAN_POINT ( 'NONE',  ( -91.79204827701150293, -283.0513426822056999, -319.2446967486595781 ) ) ;
#31433=CARTESIAN_POINT ( 'NONE',  ( -19.38173125664873098, -280.8216104470338337, -343.4042685941485615 ) ) ;
#31434=CARTESIAN_POINT ( 'NONE',  ( 5.727060680011258675, -275.0307334462215749, -330.0935966042761152 ) ) ;
#31435=CARTESIAN_POINT ( 'NONE',  ( 36.77616498652003685, -283.4039849914132674, -258.8089732207753855 ) ) ;
#31438=CARTESIAN_POINT ( 'NONE',  ( -1.657897437980451638, -272.9169497584712190, -203.0327685112679603 ) ) ;
#31439=CARTESIAN_POINT ( 'NONE',  ( -96.47058215272042503, -279.9167293225235653, -316.7702091354408935 ) ) ;
#31441=CARTESIAN_POINT ( 'NONE',  ( -66.65344565458198645, -287.5913188514035710, -200.7182018045904499 ) ) ;
#31443=CARTESIAN_POINT ( 'NONE',  ( -71.80289454216593015, -289.5965874161616966, -203.7329695588857987 ) ) ;
#31445=CARTESIAN_POINT ( 'NONE',  ( -109.1645180587833721, -295.5462285602326347, -255.1807846526926085 ) ) ;
#31446=CARTESIAN_POINT ( 'NONE',  ( -48.26576599665141742, -287.3320686382022586, -343.8400452356967776 ) ) ;
#31447=CARTESIAN_POINT ( 'NONE',  ( -33.93809357080956346, -124.0300793293349244, -358.8670080828285336 ) ) ;
#31448=CARTESIAN_POINT ( 'NONE',  ( -50.27442350059632048, -295.8868865789812617, -196.4845634323208685 ) ) ;
#31449=CARTESIAN_POINT ( 'NONE',  ( 22.72955719232091809, -286.6669441281401305, -317.4369254192948802 ) ) ;
#31450=CARTESIAN_POINT ( 'NONE',  ( 21.13749052054649624, -282.5253132608652322, -225.3225386360151674 ) ) ;
#31451=CARTESIAN_POINT ( 'NONE',  ( -80.99794473902790060, -281.8754884775376013, -332.6192447034292741 ) ) ;
#31452=CARTESIAN_POINT ( 'NONE',  ( -87.93059018348077416, -291.3209759682179651, -217.6627103320107892 ) ) ;
#31453=CARTESIAN_POINT ( 'NONE',  ( 21.49183279404825697, -283.5933680662857910, -314.5859102448242766 ) ) ;
#31454=CARTESIAN_POINT ( 'NONE',  ( 12.03317942220703785, -283.1470862150221706, -324.3492925763025596 ) ) ;
#31455=CARTESIAN_POINT ( 'NONE',  ( -74.82320468229929133, -291.5285159201268925, -335.7334639684534068 ) ) ;
#31456=CARTESIAN_POINT ( 'NONE',  ( -111.0181294507624870, -273.1675587053790082, -247.8735358820989916 ) ) ;
#31458=CARTESIAN_POINT ( 'NONE',  ( -59.62635283859822266, -287.4184195001796525, -342.5602069620944121 ) ) ;
#31459=CARTESIAN_POINT ( 'NONE',  ( 36.88562052154607329, -275.8092279621046714, -290.8872163294952315 ) ) ;
#31460=CARTESIAN_POINT ( 'NONE',  ( 27.65462333698635078, -295.0394239356660933, -233.5497195466952576 ) ) ;
#31462=CARTESIAN_POINT ( 'NONE',  ( -69.91165696735023971, -288.1233781216987495, -202.8022627189028810 ) ) ;
#31464=ADVANCED_FACE ( 'NONE', ( #25691 ), #81887, .F. ) ;
#31466=CARTESIAN_POINT ( 'NONE',  ( -34.06901696572148808, -296.4923565346082910, -194.1619862224283963 ) ) ;
#31467=CARTESIAN_POINT ( 'NONE',  ( -32.12080932589464055, -293.7192026483698442, -196.7332609505925802 ) ) ;
#31468=CARTESIAN_POINT ( 'NONE',  ( -14.02508717325673615, -273.7113827915954971, -201.0774386031104086 ) ) ;
#31469=CARTESIAN_POINT ( 'NONE',  ( -90.32816228578657558, -292.8053666004113325, -219.1444939209810059 ) ) ;
#31470=CARTESIAN_POINT ( 'NONE',  ( -81.88161658258529485, -292.3697966766944205, -212.1625740438936134 ) ) ;
#31471=CARTESIAN_POINT ( 'NONE',  ( -84.30796038583113727, -287.1562652393751023, -213.0918503038076892 ) ) ;
#31472=CARTESIAN_POINT ( 'NONE',  ( -50.48299935605892585, -293.3127650641675359, -195.0888618316279235 ) ) ;
#31473=CARTESIAN_POINT ( 'NONE',  ( -86.21098281291396859, -292.7060542423684524, -211.4272894462813213 ) ) ;
#31474=CARTESIAN_POINT ( 'NONE',  ( -20.85023846380252621, -294.6679889053587544, -341.5260319559981781 ) ) ;
#31475=CARTESIAN_POINT ( 'NONE',  ( 23.60226443846766387, -288.9565606166154339, -226.5605124199157103 ) ) ;
#31476=CARTESIAN_POINT ( 'NONE',  ( 25.10853272907954192, -282.3163307100768975, -315.4275724825068323 ) ) ;
#31477=CARTESIAN_POINT ( 'NONE',  ( -90.60283952281481845, -295.3843222647720950, -216.7648006912653500 ) ) ;
#31478=CARTESIAN_POINT ( 'NONE',  ( -114.3265517440705850, -284.4261035551376153, -267.1122898648237083 ) ) ;
#31479=CARTESIAN_POINT ( 'NONE',  ( 32.81615884907151326, -277.8659331739482923, -296.0011001146751823 ) ) ;
#31480=CARTESIAN_POINT ( 'NONE',  ( -94.60438968308704943, -282.7015653039973131, -316.2953292274448245 ) ) ;
#31481=CARTESIAN_POINT ( 'NONE',  ( 14.92417007275667906, -284.7889119931800792, -216.5719047580091967 ) ) ;
#31482=CARTESIAN_POINT ( 'NONE',  ( -31.56841561323425793, -275.1197215282965658, -345.9574184079501720 ) ) ;
#31484=CARTESIAN_POINT ( 'NONE',  ( -95.97487510789744647, -283.4488949960186233, -313.9517045076565864 ) ) ;
#31485=CARTESIAN_POINT ( 'NONE',  ( -110.9599172156418234, -280.0240787768369159, -249.1864436785759835 ) ) ;
#31486=CARTESIAN_POINT ( 'NONE',  ( 22.81500075064044708, -285.9706276463091967, -222.6537746429988545 ) ) ;
#31487=CARTESIAN_POINT ( 'NONE',  ( 30.42676385983788734, -295.7071143573116956, -300.1169459792799330 ) ) ;
#31488=CARTESIAN_POINT ( 'NONE',  ( -25.87008381219308717, -278.5084972166658872, -345.6926680327092640 ) ) ;
#31489=CARTESIAN_POINT ( 'NONE',  ( 39.13128916600017959, -276.9131735701977846, -274.0036748556526618 ) ) ;
#31490=CARTESIAN_POINT ( 'NONE',  ( -32.42267914001488549, -276.8218678416092757, -343.2451645309615174 ) ) ;
#31491=CARTESIAN_POINT ( 'NONE',  ( -80.81323830243850637, -299.4608118150424048, -209.4492653379770104 ) ) ;
#31492=CARTESIAN_POINT ( 'NONE',  ( 35.47938801786849439, -285.7738233037552504, -287.5982161197611049 ) ) ;
#31493=CARTESIAN_POINT ( 'NONE',  ( -109.6779848185424271, -292.4588604657840847, -246.2395989081465757 ) ) ;
#31494=CARTESIAN_POINT ( 'NONE',  ( 12.55524525566281824, -293.2576136460835414, -324.1384175559534810 ) ) ;
#31496=CARTESIAN_POINT ( 'NONE',  ( 33.66932302133138677, -292.9938145533351417, -253.2923385062885302 ) ) ;
#31498=CARTESIAN_POINT ( 'NONE',  ( -17.78981403259718519, -289.8853875712802051, -344.5178186846274571 ) ) ;
#31499=CARTESIAN_POINT ( 'NONE',  ( -99.55884111655753088, -279.7331790903643878, -231.8858920068892928 ) ) ;
#31500=CARTESIAN_POINT ( 'NONE',  ( -110.5140328788520208, -295.7641767339590615, -247.2221190868052076 ) ) ;
#31501=CARTESIAN_POINT ( 'NONE',  ( 16.22223479531319512, -287.4400584448364953, -215.1866885617002083 ) ) ;
#31502=CARTESIAN_POINT ( 'NONE',  ( -36.08293038156391930, -289.3700871971960851, -347.3427883231039459 ) ) ;
#31504=CARTESIAN_POINT ( 'NONE',  ( -71.41498665744305185, -283.8485688112849630, -334.9451611505753590 ) ) ;
#31505=CARTESIAN_POINT ( 'NONE',  ( 185.1013737608651013, 263.7048346170037689, -153.2992251502632541 ) ) ;
#31506=CARTESIAN_POINT ( 'NONE',  ( 137.2480117259403585, 180.4972570205891884, -240.1171119101352360 ) ) ;
#31507=CARTESIAN_POINT ( 'NONE',  ( 198.0687835817796270, 286.2794921413739644, -96.29896154386530327 ) ) ;
#31508=CARTESIAN_POINT ( 'NONE',  ( -5.003894491223660701, -275.8123695864867955, -336.0017711361109605 ) ) ;
#31509=CARTESIAN_POINT ( 'NONE',  ( -106.5606084506377158, -277.1508379602009313, -294.6599019257305372 ) ) ;
#31510=CARTESIAN_POINT ( 'NONE',  ( -96.00881876065979270, -272.8911064653503900, -220.5019487167899683 ) ) ;
#31511=CARTESIAN_POINT ( 'NONE',  ( -20.25196880903670760, -109.6380444505058875, -360.0496258023737255 ) ) ;
#31512=CARTESIAN_POINT ( 'NONE',  ( -45.61305577217230933, -275.8395903467039147, -346.4722550337872349 ) ) ;
#31514=CARTESIAN_POINT ( 'NONE',  ( -102.8978902630445162, -290.6078008813500446, -302.6159529138357129 ) ) ;
#31515=CARTESIAN_POINT ( 'NONE',  ( -73.21436098207674092, -298.3920489143060877, -202.3515921096798991 ) ) ;
#31516=CARTESIAN_POINT ( 'NONE',  ( 35.76666439674846742, -286.1385583460980229, -262.8504246756956491 ) ) ;
#31517=CARTESIAN_POINT ( 'NONE',  ( -73.90372298529642592, -274.2314020529892673, -202.6518564366450619 ) ) ;
#31518=CARTESIAN_POINT ( 'NONE',  ( -7.986360240581060310, -294.8232467900217557, -337.2122899830308143 ) ) ;
#31520=CARTESIAN_POINT ( 'NONE',  ( -39.88943947318689709, -279.0040441156530164, -345.8909794018489379 ) ) ;
#31521=CARTESIAN_POINT ( 'NONE',  ( 37.13066177362677678, -281.3018527613390347, -289.6845290741199506 ) ) ;
#31522=CARTESIAN_POINT ( 'NONE',  ( -104.5492971991351396, -279.2382614340767191, -299.7690583863771394 ) ) ;
#31523=CARTESIAN_POINT ( 'NONE',  ( -111.1850398229012029, -280.0844894610270899, -288.3357977039410684 ) ) ;
#31524=CARTESIAN_POINT ( 'NONE',  ( -35.10724925903871707, -296.6553866802951802, -196.7724395101816697 ) ) ;
#31526=CARTESIAN_POINT ( 'NONE',  ( -19.53660966853966130, -280.4541412895488293, -199.5134983381287839 ) ) ;
#31527=CARTESIAN_POINT ( 'NONE',  ( 9.403993259544019878, -275.4793498521829065, -209.3775220758666080 ) ) ;
#31529=CARTESIAN_POINT ( 'NONE',  ( -49.42284890972417344, -275.8984366434439721, -196.2881265882443245 ) ) ;
#31530=CARTESIAN_POINT ( 'NONE',  ( -9.443979966876431931, -275.2693160853962695, -341.4970688285294500 ) ) ;
#31532=CARTESIAN_POINT ( 'NONE',  ( -109.4340990374851827, -289.9171451653010081, -257.6106457475736420 ) ) ;
#31533=CARTESIAN_POINT ( 'NONE',  ( -105.3380788153204861, -284.3663475748666656, -234.3332694592615724 ) ) ;
#31534=CARTESIAN_POINT ( 'NONE',  ( 36.36364369795897034, -279.6971856230323965, -263.0735535312934985 ) ) ;
#31535=CARTESIAN_POINT ( 'NONE',  ( 34.64537128652856524, -279.9262687849906115, -255.0289241323234251 ) ) ;
#31536=CARTESIAN_POINT ( 'NONE',  ( -102.2348916860821362, -283.1226445814353383, -233.7838005970184554 ) ) ;
#31537=CARTESIAN_POINT ( 'NONE',  ( -105.9124871877583587, -292.1528278534239007, -300.8691199131528151 ) ) ;
#31538=CARTESIAN_POINT ( 'NONE',  ( -7.853927069331436250, -281.6524336797021419, -203.1342657585906295 ) ) ;
#31540=CARTESIAN_POINT ( 'NONE',  ( 6.448440001255717036, -280.8683752031685117, -332.7863864229117326 ) ) ;
#31541=CARTESIAN_POINT ( 'NONE',  ( 20.75402089830514640, -296.2061393517508350, -317.8142709803955199 ) ) ;
#31542=CARTESIAN_POINT ( 'NONE',  ( -110.3572456723334625, -277.0593407210012629, -249.3205827328843895 ) ) ;
#31543=CARTESIAN_POINT ( 'NONE',  ( -26.90155557060899127, -288.1846429851541984, -195.8707869940245132 ) ) ;
#31545=CARTESIAN_POINT ( 'NONE',  ( -85.61225569124820822, -293.3109369479820430, -212.1616937219453121 ) ) ;
#31546=CARTESIAN_POINT ( 'NONE',  ( 18.91909998922363201, -274.2415484314500986, -319.9760793501604326 ) ) ;
#31547=CARTESIAN_POINT ( 'NONE',  ( -15.00897166139726835, -287.9673546918364764, -343.9382301464443685 ) ) ;
#31548=CARTESIAN_POINT ( 'NONE',  ( -37.53177539934910811, -290.4496402685245471, -196.5487794936665011 ) ) ;
#31550=CARTESIAN_POINT ( 'NONE',  ( -7.321431726798665274, -275.3347851384361888, -337.4433582877732647 ) ) ;
#31551=CARTESIAN_POINT ( 'NONE',  ( -53.43993691015518266, -293.4002685872633833, -342.8826839796104764 ) ) ;
#31552=CARTESIAN_POINT ( 'NONE',  ( -97.74473777446802103, -291.2876605789508062, -312.2486780554531265 ) ) ;
#31555=CARTESIAN_POINT ( 'NONE',  ( 8.450459310464765394, -291.1459038160550676, -209.2559432353779414 ) ) ;
#31556=CARTESIAN_POINT ( 'NONE',  ( 26.39715891917249024, -289.6585161460777726, -307.6616315402754367 ) ) ;
#31557=CARTESIAN_POINT ( 'NONE',  ( -62.45024806280846263, -287.6141186812323554, -342.1352080013635373 ) ) ;
#31558=CARTESIAN_POINT ( 'NONE',  ( -19.69197021346174736, -287.7088607427220950, -198.9197997599313226 ) ) ;
#31559=CARTESIAN_POINT ( 'NONE',  ( 82.64890176555634582, -299.5541904835127980, -195.3611179825600175 ) ) ;
#31560=CARTESIAN_POINT ( 'NONE',  ( 27.17768217025705368, -288.8254375019553208, -304.9631865892729934 ) ) ;
#31561=CARTESIAN_POINT ( 'NONE',  ( -68.81741396434107116, -297.4437433937206379, -338.8419199787858247 ) ) ;
#31564=CARTESIAN_POINT ( 'NONE',  ( 16.01157806488294355, -287.9936317547674776, -215.3935236749062199 ) ) ;
#31565=CARTESIAN_POINT ( 'NONE',  ( -73.43100056112321283, -275.6068397501877598, -336.7601514665065565 ) ) ;
#31566=CARTESIAN_POINT ( 'NONE',  ( -84.84999387199226817, -278.0199904630671313, -330.9986935340729701 ) ) ;
#31568=CARTESIAN_POINT ( 'NONE',  ( -62.03682781304478056, -279.4065165195858071, -197.3947179004950669 ) ) ;
#31569=CARTESIAN_POINT ( 'NONE',  ( -36.48437828106663261, -300.0428251152431471, -195.7160183634054533 ) ) ;
#31570=CARTESIAN_POINT ( 'NONE',  ( -80.43826238227499914, -283.4684023602599154, -208.9158880382875338 ) ) ;
#31572=CARTESIAN_POINT ( 'NONE',  ( -65.25903034396264957, -277.8229345540986515, -201.5753043661879644 ) ) ;
#31574=CARTESIAN_POINT ( 'NONE',  ( -16.71693364395909498, -280.7856996563839402, -342.5233499504229826 ) ) ;
#31576=CARTESIAN_POINT ( 'NONE',  ( -1.807912934046726150, -275.0699185338702932, -337.8893174391120624 ) ) ;
#31577=CARTESIAN_POINT ( 'NONE',  ( -82.77216404776073944, -297.2060057020833028, -328.4501323682479210 ) ) ;
#31578=CARTESIAN_POINT ( 'NONE',  ( -10.82188127496737629, -281.6347668122014056, -342.3771860588033178 ) ) ;
#31579=CARTESIAN_POINT ( 'NONE',  ( -77.65145518012722903, -298.4379283258955411, -209.1566359537868323 ) ) ;
#31580=CARTESIAN_POINT ( 'NONE',  ( -73.06536452449314822, -298.9043072148883198, -202.6482391785336006 ) ) ;
#31581=CARTESIAN_POINT ( 'NONE',  ( -6.516195927483879657, -274.1352291704450863, -204.1653796178599407 ) ) ;
#31582=CARTESIAN_POINT ( 'NONE',  ( 35.72962495944016581, -295.7699498266229625, -287.3169562006386286 ) ) ;
#31583=CARTESIAN_POINT ( 'NONE',  ( 39.60443700471466144, -287.7696040085465370, -274.4208188855158710 ) ) ;
#31584=CARTESIAN_POINT ( 'NONE',  ( -61.56244935526919448, -277.8198993089526994, -198.7331171753913281 ) ) ;
#31585=CARTESIAN_POINT ( 'NONE',  ( -80.54236993324256844, -289.4532246197836116, -334.1648610695394268 ) ) ;
#31586=CARTESIAN_POINT ( 'NONE',  ( -99.04644691724929828, -289.0670534464729826, -309.8064303995699333 ) ) ;
#31587=CARTESIAN_POINT ( 'NONE',  ( -4.182043124565208103, -290.4891287363078618, -203.0755806985293361 ) ) ;
#31589=CARTESIAN_POINT ( 'NONE',  ( -111.8441652935849646, -278.1196860901031300, -270.4320060261264871 ) ) ;
#31590=CARTESIAN_POINT ( 'NONE',  ( 30.54003665176527349, -287.4226542853485284, -297.5171275647541620 ) ) ;
#31592=CARTESIAN_POINT ( 'NONE',  ( -114.1055335641777617, -285.4979963134953778, -269.9949370531536488 ) ) ;
#31593=CARTESIAN_POINT ( 'NONE',  ( -27.86621114069169280, -291.2282787155681376, -194.1299505027877501 ) ) ;
#31594=CARTESIAN_POINT ( 'NONE',  ( 19.42890481214846687, -283.5688955815255099, -321.7260395084860534 ) ) ;
#31595=CARTESIAN_POINT ( 'NONE',  ( 3.388460919053434051, -282.3213103595576854, -331.0032326712681652 ) ) ;
#31596=CARTESIAN_POINT ( 'NONE',  ( -114.3379633736027046, -296.5616392792451848, -269.6025362622565922 ) ) ;
#31597=CARTESIAN_POINT ( 'NONE',  ( 24.40777402064800938, -277.4164340614624962, -310.3077885963562039 ) ) ;
#31598=CARTESIAN_POINT ( 'NONE',  ( -65.93419239661774611, -289.6963316534138357, -201.3957521531118005 ) ) ;
#31599=CARTESIAN_POINT ( 'NONE',  ( 33.24612186818926318, -274.0804437606964825, -250.0674406358796489 ) ) ;
#31602=CARTESIAN_POINT ( 'NONE',  ( 5.535221885216643045, -288.5575120494830799, -209.4467284744862070 ) ) ;
#31603=CARTESIAN_POINT ( 'NONE',  ( -36.26494212304582732, -296.1186519479138610, -347.0574989538328055 ) ) ;
#31604=CARTESIAN_POINT ( 'NONE',  ( -108.1899705745931044, -284.9661675174141351, -288.3726488235844272 ) ) ;
#31605=CARTESIAN_POINT ( 'NONE',  ( 19.69432321872898584, -275.3106535725914341, -321.7589162018619504 ) ) ;
#31606=CARTESIAN_POINT ( 'NONE',  ( 4.079631519686741647, -293.2456110996500911, -205.5092249541860099 ) ) ;
#31607=CARTESIAN_POINT ( 'NONE',  ( 36.18396607520516994, -285.4592748441824597, -252.0777404733550213 ) ) ;
#31608=CARTESIAN_POINT ( 'NONE',  ( 39.69045920771608138, -293.8847398970609106, -270.3057362904817182 ) ) ;
#31609=CARTESIAN_POINT ( 'NONE',  ( -109.9943504101857314, -290.9820580472552365, -263.0344616019719979 ) ) ;
#31610=CARTESIAN_POINT ( 'NONE',  ( 128.9467878515196162, -299.5541904835127980, -201.6105732245967488 ) ) ;
#31612=CARTESIAN_POINT ( 'NONE',  ( -76.41338813104214012, -208.2854332698812243, -353.5099304025617357 ) ) ;
#31613=CARTESIAN_POINT ( 'NONE',  ( -109.5621785376481512, -285.7590397302182623, -294.9966664917826051 ) ) ;
#31614=CARTESIAN_POINT ( 'NONE',  ( 40.64545035920995986, -273.2666405000204009, -288.1938231032136741 ) ) ;
#31616=CARTESIAN_POINT ( 'NONE',  ( -56.41250293446099562, -282.2240861343788083, -341.1462191906463772 ) ) ;
#31617=CARTESIAN_POINT ( 'NONE',  ( -89.20100201988842059, -277.4252228645872265, -327.2501072400982025 ) ) ;
#31618=CARTESIAN_POINT ( 'NONE',  ( 36.96326303731531482, -283.6719962765264427, -279.6614286388080473 ) ) ;
#31619=CARTESIAN_POINT ( 'NONE',  ( -105.1058646074189653, -262.8840186013622429, -316.9941098723735990 ) ) ;
#31620=CARTESIAN_POINT ( 'NONE',  ( -71.49181066764296588, -282.0691204901697802, -338.7159001505358447 ) ) ;
#31621=CARTESIAN_POINT ( 'NONE',  ( 35.61298303957731548, -285.7767479664731241, -286.2153042961209053 ) ) ;
#31622=CARTESIAN_POINT ( 'NONE',  ( -89.33275675203243793, -275.1903692999144937, -215.1783313827606605 ) ) ;
#31623=CARTESIAN_POINT ( 'NONE',  ( -3.109377626976773890, -295.0793128955564839, -334.9067339296058208 ) ) ;
#31624=CARTESIAN_POINT ( 'NONE',  ( -32.10554565368732227, -290.8043708015716220, -197.0420268373906083 ) ) ;
#31625=CARTESIAN_POINT ( 'NONE',  ( -103.5138418283205937, -278.6913751229081413, -309.6389870895413878 ) ) ;
#31626=CARTESIAN_POINT ( 'NONE',  ( 33.24219355772338247, -275.7980969960622701, -288.9867442042744301 ) ) ;
#31627=CARTESIAN_POINT ( 'NONE',  ( 36.29296320578048096, -274.2004955341757295, -248.7411298974482463 ) ) ;
#31629=CARTESIAN_POINT ( 'NONE',  ( -33.69173762154775886, -275.0060845995964200, -345.2849583103067062 ) ) ;
#31630=CARTESIAN_POINT ( 'NONE',  ( 32.88227782188145909, -295.3655190961599146, -300.6145655306884237 ) ) ;
#31634=CARTESIAN_POINT ( 'NONE',  ( -87.12872584445554480, -284.8447281865615537, -324.2402024237510432 ) ) ;
#31635=CARTESIAN_POINT ( 'NONE',  ( -70.01382348071287254, -285.2366746354434213, -338.9793698795769501 ) ) ;
#31636=CARTESIAN_POINT ( 'NONE',  ( -68.81131046605683821, -284.9757417579568255, -204.3658256840728598 ) ) ;
#31637=CARTESIAN_POINT ( 'NONE',  ( -64.64789361071770202, -275.8144449706422279, -338.9778654478266731 ) ) ;
#31638=CARTESIAN_POINT ( 'NONE',  ( 36.36915669432283238, -283.5322742621667658, -279.5886563088085381 ) ) ;
#31639=CARTESIAN_POINT ( 'NONE',  ( -13.57998123185541850, -275.2180122261977431, -340.1721088107518085 ) ) ;
#31640=CARTESIAN_POINT ( 'NONE',  ( -78.79551492306752891, -278.7047127963085700, -330.8861960760188481 ) ) ;
#31642=CARTESIAN_POINT ( 'NONE',  ( -95.78964758816373148, -280.0293439850141795, -220.4610873726086027 ) ) ;
#31643=CARTESIAN_POINT ( 'NONE',  ( -22.58413131596649848, -280.7284065665521098, -194.7970326231106526 ) ) ;
#31647=CARTESIAN_POINT ( 'NONE',  ( 36.30936625334612700, -289.6391041640442268, -288.1874893336914170 ) ) ;
#31648=CARTESIAN_POINT ( 'NONE',  ( -108.4583930955421636, -295.5225415981411743, -287.5900575030865411 ) ) ;
#31649=CARTESIAN_POINT ( 'NONE',  ( -107.1643914186132918, -290.3148879563284481, -238.0146506444686736 ) ) ;
#31650=CARTESIAN_POINT ( 'NONE',  ( 35.56953862388974130, -285.6226743145971341, -257.3465426152315558 ) ) ;
#31651=CARTESIAN_POINT ( 'NONE',  ( -27.74185880043491537, -284.7511786946188863, -197.4007317255870078 ) ) ;
#31652=CARTESIAN_POINT ( 'NONE',  ( -107.5251792754394558, -289.0998521598905313, -246.8610484537966272 ) ) ;
#31653=CARTESIAN_POINT ( 'NONE',  ( -46.79111464945430043, -287.1347290993908814, -197.5238096685875462 ) ) ;
#31654=CARTESIAN_POINT ( 'NONE',  ( -7.254749641371684099, -287.0639612120409652, -340.3838921088807865 ) ) ;
#31655=CARTESIAN_POINT ( 'NONE',  ( 6.357400499688796280, -288.6453714808767472, -209.3431758782986662 ) ) ;
#31656=CARTESIAN_POINT ( 'NONE',  ( -18.21598123060010721, -286.8060514119883919, -343.0538638398181774 ) ) ;
#31657=CARTESIAN_POINT ( 'NONE',  ( -40.23168218731265000, -284.0306225597175285, -343.5393692074190994 ) ) ;
#31658=CARTESIAN_POINT ( 'NONE',  ( -109.0255577970418415, -292.2592061426248051, -293.1462992156468772 ) ) ;
#31659=CARTESIAN_POINT ( 'NONE',  ( 82.12709634636649980, -301.2636011320335570, -194.3234711915518460 ) ) ;
#31661=CARTESIAN_POINT ( 'NONE',  ( -84.34020419986087802, -299.3312816093250035, -211.1964764290941901 ) ) ;
#31662=CARTESIAN_POINT ( 'NONE',  ( -6.692461502728587419, -279.6622820339377995, -203.9153265435139986 ) ) ;
#31663=CARTESIAN_POINT ( 'NONE',  ( 23.75719899250687916, -278.9606242146725208, -226.8648517451182443 ) ) ;
#31664=CARTESIAN_POINT ( 'NONE',  ( -3.309518236176309358, -293.8114320374659201, -339.2666871655222849 ) ) ;
#31665=CARTESIAN_POINT ( 'NONE',  ( -88.01092423530337783, -271.5719422238865945, -216.3409571816720245 ) ) ;
#31666=CARTESIAN_POINT ( 'NONE',  ( 35.29306575426716819, -273.8435390795626176, -286.7133208401646129 ) ) ;
#31667=CARTESIAN_POINT ( 'NONE',  ( -104.3796268654500210, -297.4628492996155842, -300.6045490638873616 ) ) ;
#31669=CARTESIAN_POINT ( 'NONE',  ( 75.13442338291717704, -297.9159792440862020, -194.0828677818368817 ) ) ;
#31670=CARTESIAN_POINT ( 'NONE',  ( -34.90982439382034386, -293.2618594751951946, -346.3088631521420098 ) ) ;
#31671=CARTESIAN_POINT ( 'NONE',  ( -57.83630956907590104, -293.2076400547692288, -199.6300493939702960 ) ) ;
#31674=CARTESIAN_POINT ( 'NONE',  ( 34.22767131610815738, -294.5555833536576529, -285.6010639303100334 ) ) ;
#31676=CARTESIAN_POINT ( 'NONE',  ( -67.25218036032539715, -281.4625194063139588, -339.5259210065718207 ) ) ;
#31677=CARTESIAN_POINT ( 'NONE',  ( 18.83309724950744624, -294.2133679068970196, -316.9807719879989918 ) ) ;
#31678=CARTESIAN_POINT ( 'NONE',  ( -67.88135284565001371, -283.4420916149674099, -341.0458377732636563 ) ) ;
#31679=CARTESIAN_POINT ( 'NONE',  ( 34.79356488540131664, -283.1843735584628234, -247.8707258188076992 ) ) ;
#31680=CARTESIAN_POINT ( 'NONE',  ( -112.3381687415402155, -284.4360108815233730, -253.0038720263462722 ) ) ;
#31681=CARTESIAN_POINT ( 'NONE',  ( -68.54293615403442175, -289.6410736254920266, -202.3285784733186574 ) ) ;
#31683=CARTESIAN_POINT ( 'NONE',  ( 15.26144635241925229, -280.8051034806416624, -325.6387511792363512 ) ) ;
#31684=CARTESIAN_POINT ( 'NONE',  ( 17.26820761434590068, -285.5373138461500275, -221.1589798619104670 ) ) ;
#31685=CARTESIAN_POINT ( 'NONE',  ( 32.57740277810245999, -286.8765904871625025, -301.8700303358252768 ) ) ;
#31686=CARTESIAN_POINT ( 'NONE',  ( -53.30275703964352374, -296.8602561139885552, -342.4670182210999769 ) ) ;
#31687=CARTESIAN_POINT ( 'NONE',  ( -112.1444856307785614, -280.1747292922206611, -254.7046915513597867 ) ) ;
#31688=CARTESIAN_POINT ( 'NONE',  ( -5.226898591084080614, -292.6517535143096325, -338.5445237236838238 ) ) ;
#31689=CARTESIAN_POINT ( 'NONE',  ( -59.73608192447613874, -279.4207704095745157, -200.8054307858841412 ) ) ;
#31690=CARTESIAN_POINT ( 'NONE',  ( 22.20790884732915771, -293.0633223826307017, -221.5467340838717973 ) ) ;
#31691=CARTESIAN_POINT ( 'NONE',  ( -112.9006632345497394, -282.6370507681265849, -269.9645206891372027 ) ) ;
#31693=CARTESIAN_POINT ( 'NONE',  ( -95.48725449159030632, -279.8994201392774244, -317.7531029649275638 ) ) ;
#31695=CARTESIAN_POINT ( 'NONE',  ( -37.00647208094338936, -294.1065667860947315, -343.6081098213658152 ) ) ;
#31696=CARTESIAN_POINT ( 'NONE',  ( -56.84443915194403729, -295.8006349699807629, -197.8873670510351985 ) ) ;
#31699=CARTESIAN_POINT ( 'NONE',  ( -13.81382168236735453, -282.3387376185723951, -199.4666214804129538 ) ) ;
#31700=CARTESIAN_POINT ( 'NONE',  ( 32.80750523410983988, -293.3302592988459310, -290.8285448946089673 ) ) ;
#31702=CARTESIAN_POINT ( 'NONE',  ( 31.98288692825983404, -272.6237833571632905, -237.0123917617631264 ) ) ;
#31703=CARTESIAN_POINT ( 'NONE',  ( -48.92262123649869210, -296.9669618639499049, -194.4215012050215705 ) ) ;
#31704=CARTESIAN_POINT ( 'NONE',  ( 18.29774641103156796, -289.5890328478654396, -322.8734999650166628 ) ) ;
#31705=CARTESIAN_POINT ( 'NONE',  ( -31.87347319535359347, -288.8146914552878570, -343.2066483003274016 ) ) ;
#31707=CARTESIAN_POINT ( 'NONE',  ( -101.4241730879958254, -280.5659399149620299, -233.9723228616421977 ) ) ;
#31708=CARTESIAN_POINT ( 'NONE',  ( -67.24908155059992509, -299.4146921300625195, -202.6455285206034773 ) ) ;
#31709=CARTESIAN_POINT ( 'NONE',  ( -9.080349657951865439, -279.2250951291436536, -202.6231923054262438 ) ) ;
#31711=CARTESIAN_POINT ( 'NONE',  ( -75.76566857880099803, -297.2209533044920704, -203.5965486413334986 ) ) ;
#31712=CARTESIAN_POINT ( 'NONE',  ( -64.62165223510481837, -293.6133828685094613, -201.0860827745362371 ) ) ;
#31714=CARTESIAN_POINT ( 'NONE',  ( -93.52349448395433740, -291.8663853719565395, -223.5708705120093782 ) ) ;
#31717=CARTESIAN_POINT ( 'NONE',  ( -40.55591917488535358, -290.1517546168335002, -194.6515535156463841 ) ) ;
#31718=CARTESIAN_POINT ( 'NONE',  ( -107.2535800384607683, -272.3426188741493092, -248.9671800270169228 ) ) ;
#31721=CARTESIAN_POINT ( 'NONE',  ( -105.3946199326761359, -292.5220187246089836, -235.7263304947500444 ) ) ;
#31722=CARTESIAN_POINT ( 'NONE',  ( -88.47809603358389552, -286.1948066931273615, -334.5364918783848793 ) ) ;
#31723=CARTESIAN_POINT ( 'NONE',  ( -7.547864174331647469, -288.4438165807034125, -201.7145174248215653 ) ) ;
#31724=CARTESIAN_POINT ( 'NONE',  ( 34.65490009692324946, -273.8157396209811623, -290.8167259753296889 ) ) ;
#31725=CARTESIAN_POINT ( 'NONE',  ( 33.42323654118416698, -277.1697606067490369, -247.0948632554170104 ) ) ;
#31726=CARTESIAN_POINT ( 'NONE',  ( -2.949643699780619688, -290.5902078109149329, -204.3421763437440575 ) ) ;
#31727=CARTESIAN_POINT ( 'NONE',  ( -31.19793442991275612, -281.9892563525241940, -194.7939784165786250 ) ) ;
#31729=CARTESIAN_POINT ( 'NONE',  ( -18.71766321217296181, -282.1546293932814820, -341.1033233331066867 ) ) ;
#31730=CARTESIAN_POINT ( 'NONE',  ( -104.6975156503065847, -279.1553599703948976, -307.0310869529659499 ) ) ;
#31731=CARTESIAN_POINT ( 'NONE',  ( -2.556667356714538819, -279.2967692811753295, -202.0968480614500891 ) ) ;
#31732=CARTESIAN_POINT ( 'NONE',  ( 63.58840756535673222, 47.24236442185751628, -315.7359544152388366 ) ) ;
#31733=CARTESIAN_POINT ( 'NONE',  ( 37.67829887599565808, -276.6983139779528642, -286.6958664055291024 ) ) ;
#31735=CARTESIAN_POINT ( 'NONE',  ( -73.63234562624435853, -275.0999704676132183, -203.1778854431856303 ) ) ;
#31736=CARTESIAN_POINT ( 'NONE',  ( -107.3452863284742449, -275.1604526064901393, -262.5058405983616012 ) ) ;
#31738=CARTESIAN_POINT ( 'NONE',  ( -73.68631503275130967, -290.6263995946848695, -334.0410824891840207 ) ) ;
#31739=CARTESIAN_POINT ( 'NONE',  ( -104.2529272901706179, -291.8404560376891368, -306.3730839265644477 ) ) ;
#31740=CARTESIAN_POINT ( 'NONE',  ( -4.780232890902527565, -291.8412761275359344, -204.8976238329101420 ) ) ;
#31741=CARTESIAN_POINT ( 'NONE',  ( -18.19127754818147125, -285.8000810026210274, -195.7890253703707799 ) ) ;
#31743=CARTESIAN_POINT ( 'NONE',  ( -37.56316512000142893, -281.4548757140970565, -344.1733544659482504 ) ) ;
#31744=CARTESIAN_POINT ( 'NONE',  ( 22.17779627711555079, -290.0249118884566428, -314.7478766808773116 ) ) ;
#31745=CARTESIAN_POINT ( 'NONE',  ( -6.985395507497001333, -281.1263059000270346, -337.5255556735269238 ) ) ;
#31746=CARTESIAN_POINT ( 'NONE',  ( 18.32719162700897542, -282.1883334674241723, -222.3603717562722011 ) ) ;
#31748=CARTESIAN_POINT ( 'NONE',  ( 38.55113162583872821, -288.3475780284512098, -258.7368638129711371 ) ) ;
#31749=CARTESIAN_POINT ( 'NONE',  ( -110.2292480326194521, -278.9689932649845332, -276.0899462611741342 ) ) ;
#31750=CARTESIAN_POINT ( 'NONE',  ( -30.71623702496241748, -290.9289376234380029, -193.9927621085660689 ) ) ;
#31751=CARTESIAN_POINT ( 'NONE',  ( 33.70620831435992670, -287.9807511608051982, -240.9586434013265830 ) ) ;
#31752=CARTESIAN_POINT ( 'NONE',  ( -3.522066819966669815, -286.9789546031654481, -201.2397336393281080 ) ) ;
#31753=CARTESIAN_POINT ( 'NONE',  ( -103.0117370278437221, -284.2858308864481387, -302.3589568781726484 ) ) ;
#31756=CARTESIAN_POINT ( 'NONE',  ( -8.995689436432197539, -294.2793800456232702, -200.0986873452157226 ) ) ;
#31757=CARTESIAN_POINT ( 'NONE',  ( 36.61024445866254950, -291.9893659132109747, -250.7042011461205107 ) ) ;
#31758=CARTESIAN_POINT ( 'NONE',  ( 17.60384876144849287, -275.3002858623294173, -318.7989869804835621 ) ) ;
#31759=CARTESIAN_POINT ( 'NONE',  ( -113.4996495248957586, -296.0352185049387685, -259.6226531438382494 ) ) ;
#31761=CARTESIAN_POINT ( 'NONE',  ( 7.109717562458071072, -291.1501353631761049, -211.5837480527513890 ) ) ;
#31762=CARTESIAN_POINT ( 'NONE',  ( -63.41575280811702697, -295.9476800648075709, -201.0384564183853229 ) ) ;
#31763=CARTESIAN_POINT ( 'NONE',  ( -66.73711755853138072, -292.8632882122278147, -203.1075683379044676 ) ) ;
#31764=CARTESIAN_POINT ( 'NONE',  ( -5.921562004080793251, -293.5548528198679037, -204.1128396214604663 ) ) ;
#31766=CARTESIAN_POINT ( 'NONE',  ( -1.600891109880263841, -292.5794578030966591, -336.5014585808833090 ) ) ;
#31767=CARTESIAN_POINT ( 'NONE',  ( -112.2245992611167793, -298.4877883262126375, -275.3867228762755417 ) ) ;
#31768=CARTESIAN_POINT ( 'NONE',  ( -13.19903733447574901, -289.6719311585343348, -339.5025692339283410 ) ) ;
#31769=CARTESIAN_POINT ( 'NONE',  ( -17.76047963875726765, -278.7807243189188853, -343.1277490994326627 ) ) ;
#31770=CARTESIAN_POINT ( 'NONE',  ( -105.9963593142793599, -276.9067761242620236, -304.4591271649478017 ) ) ;
#31771=CARTESIAN_POINT ( 'NONE',  ( -95.94461552330328402, -272.5730258650728501, -220.5511780372910096 ) ) ;
#31772=CARTESIAN_POINT ( 'NONE',  ( 20.45490370165923721, -280.2831900985194693, -317.2945993183348037 ) ) ;
#31773=CARTESIAN_POINT ( 'NONE',  ( -51.18746048210949340, -275.6261829625855739, -345.2926556269869138 ) ) ;
#31775=CARTESIAN_POINT ( 'NONE',  ( -107.3441061250242825, -294.9402167524035008, -292.9069301903481914 ) ) ;
#31776=CARTESIAN_POINT ( 'NONE',  ( -94.69784351963394897, -273.8422338702360435, -225.0382155619596176 ) ) ;
#31777=CARTESIAN_POINT ( 'NONE',  ( -112.0323145975978321, -288.7047437098329965, -259.9941125139034739 ) ) ;
#31778=CARTESIAN_POINT ( 'NONE',  ( -63.30473799775171528, -273.5375915509443985, -202.1206455988851189 ) ) ;
#31779=CARTESIAN_POINT ( 'NONE',  ( -31.82677828541186216, -288.9845056599974100, -347.2159241085329882 ) ) ;
#31780=CARTESIAN_POINT ( 'NONE',  ( -56.98577446623215792, -299.7800471105067572, -197.5573270854397094 ) ) ;
#31781=CARTESIAN_POINT ( 'NONE',  ( -110.5679336986514585, -294.7512726635061995, -254.8740717498590982 ) ) ;
#31782=CARTESIAN_POINT ( 'NONE',  ( -10.76749526745584618, -281.9115609947952521, -342.5145941235296050 ) ) ;
#31784=CARTESIAN_POINT ( 'NONE',  ( 28.37792330265520846, -279.0702568186964072, -234.1169682662477385 ) ) ;
#31786=CARTESIAN_POINT ( 'NONE',  ( -110.3664153697937564, -289.4439490184408896, -262.9772525857731580 ) ) ;
#31787=CARTESIAN_POINT ( 'NONE',  ( -110.1962111355657754, -282.5068708570287868, -284.6119322945127124 ) ) ;
#31790=CARTESIAN_POINT ( 'NONE',  ( -85.08307072620955580, -289.3929332587509293, -212.5185542506116860 ) ) ;
#31791=CARTESIAN_POINT ( 'NONE',  ( -89.74871073326912096, -274.8161165442882066, -218.5517270248318482 ) ) ;
#31792=CARTESIAN_POINT ( 'NONE',  ( -70.28537121042901958, -284.6816990562390401, -339.5327396634178285 ) ) ;
#31793=CARTESIAN_POINT ( 'NONE',  ( -3.186173223533343535, -272.5795070579386561, -202.9470280987365527 ) ) ;
#31794=CARTESIAN_POINT ( 'NONE',  ( -107.7611527384710541, -284.2974269724152236, -289.6463136459557859 ) ) ;
#31795=CARTESIAN_POINT ( 'NONE',  ( 35.29170777241810697, -277.1361690703892009, -282.4916152360212891 ) ) ;
#31796=CARTESIAN_POINT ( 'NONE',  ( -56.63292713618687912, -278.1099745024274057, -340.9860351287802587 ) ) ;
#31798=CARTESIAN_POINT ( 'NONE',  ( 14.39285596943708789, -284.3248188417588835, -324.6615447973005075 ) ) ;
#31801=CARTESIAN_POINT ( 'NONE',  ( 26.51055703655141471, -293.9524580666045495, -313.3947009090193205 ) ) ;
#31802=CARTESIAN_POINT ( 'NONE',  ( 5.652619050774053910, -288.6172405577019617, -209.2787414049485619 ) ) ;
#31804=DIRECTION ( 'NONE',  ( 0.000000000000000000, 0.000000000000000000, -1.000000000000000000 ) ) ;
#31805=CARTESIAN_POINT ( 'NONE',  ( 36.57525178469694538, -291.4809262143062369, -305.9938812882205070 ) ) ;
#31806=CARTESIAN_POINT ( 'NONE',  ( -95.09618839529409229, -277.0620616649609360, -321.0422575294525132 ) ) ;
#31807=CARTESIAN_POINT ( 'NONE',  ( -30.74599173846373645, -290.5339486922550805, -194.3948969467839447 ) ) ;
#31808=CARTESIAN_POINT ( 'NONE',  ( -93.79862918966466623, -286.7385158621798382, -222.9973880291659896 ) ) ;
#31809=CARTESIAN_POINT ( 'NONE',  ( -62.10807861360017768, -279.1386519388497618, -340.1622862601814745 ) ) ;
#31810=CARTESIAN_POINT ( 'NONE',  ( -69.56104999889298313, -287.0616343506380872, -201.0610778605604878 ) ) ;
#31811=CARTESIAN_POINT ( 'NONE',  ( 22.62392511233066372, -284.1681633043053239, -315.4281530696096638 ) ) ;
#31812=CARTESIAN_POINT ( 'NONE',  ( -22.93681887511569073, -277.0395634160643112, -346.0558967817065650 ) ) ;
#31813=CARTESIAN_POINT ( 'NONE',  ( -80.22794689398779155, -277.4484990829081426, -334.3766129019576283 ) ) ;
#31814=CARTESIAN_POINT ( 'NONE',  ( -101.1433752010043747, -298.9909116034737053, -231.9116312453902822 ) ) ;
#31816=CARTESIAN_POINT ( 'NONE',  ( -95.99890600148557951, -275.6948066931273615, -223.6242672951989618 ) ) ;
#31818=CARTESIAN_POINT ( 'NONE',  ( -70.17202744168670847, -295.7637598136120687, -202.0787989412391994 ) ) ;
#31820=CARTESIAN_POINT ( 'NONE',  ( -24.32479269652457177, -276.3892560612371767, -342.3052298048591524 ) ) ;
#31821=CARTESIAN_POINT ( 'NONE',  ( -76.24436942978653065, -274.7497161139079935, -204.3104947960326854 ) ) ;
#31823=CARTESIAN_POINT ( 'NONE',  ( 30.51943510554037431, -280.1448344558133954, -234.3634104413949615 ) ) ;
#31824=CARTESIAN_POINT ( 'NONE',  ( 36.69337778888591828, -289.2849849583721493, -268.2616577575786323 ) ) ;
#31825=CARTESIAN_POINT ( 'NONE',  ( -110.5447287818828102, -297.7990780355128209, -291.9483894297014785 ) ) ;
#31826=CARTESIAN_POINT ( 'NONE',  ( -110.4163765976229428, -297.4664551539190143, -293.3854289970482796 ) ) ;
#31827=CARTESIAN_POINT ( 'NONE',  ( 19.86196082207895586, -294.8835905162221707, -222.1141532739970046 ) ) ;
#31828=CARTESIAN_POINT ( 'NONE',  ( 34.50163982809560537, -279.2817490408192498, -249.4192238045684746 ) ) ;
#31829=CARTESIAN_POINT ( 'NONE',  ( 37.14402007957295382, -283.4845641785113344, -271.3081467475175828 ) ) ;
#31830=CARTESIAN_POINT ( 'NONE',  ( -73.52587143549826010, -295.6478766138080232, -205.3071408107068407 ) ) ;
#31831=CARTESIAN_POINT ( 'NONE',  ( -106.2732027943526560, -285.7318680082088918, -302.8401628202364009 ) ) ;
#31832=CARTESIAN_POINT ( 'NONE',  ( 9.237442516738328280, -285.6300666963919070, -213.7518471595305414 ) ) ;
#31833=CARTESIAN_POINT ( 'NONE',  ( 37.88668148172862260, -280.7003687205219649, -254.3606081014471272 ) ) ;
#31834=CARTESIAN_POINT ( 'NONE',  ( 66.45820036739932846, 46.88234517766255749, -318.5738176559102044 ) ) ;
#31836=CARTESIAN_POINT ( 'NONE',  ( 22.81227569721311355, -286.7617784443814912, -317.5001754276903512 ) ) ;
#31837=CARTESIAN_POINT ( 'NONE',  ( 13.15724001548059441, -286.4481424706384018, -217.5472115923622312 ) ) ;
#31839=CARTESIAN_POINT ( 'NONE',  ( -113.8988191518282491, -285.5646572735515747, -275.7099750386934147 ) ) ;
#31840=CARTESIAN_POINT ( 'NONE',  ( 23.06743953656408053, -275.3148381989095128, -229.3164619267827788 ) ) ;
#31841=CARTESIAN_POINT ( 'NONE',  ( -33.54087841627652011, -291.0192777922545702, -193.7644714204199374 ) ) ;
#31842=CARTESIAN_POINT ( 'NONE',  ( 30.99036858264368277, -282.6588078435840430, -305.6320858171718555 ) ) ;
#31844=CARTESIAN_POINT ( 'NONE',  ( -112.3185891297875543, -280.2521489285202279, -256.1075677718598627 ) ) ;
#31845=CARTESIAN_POINT ( 'NONE',  ( 25.91537443563242959, -282.4653371581390502, -314.2509961836761363 ) ) ;
#31846=CARTESIAN_POINT ( 'NONE',  ( -92.05005921254146983, -282.6952119285918457, -226.6919474004047572 ) ) ;
#31847=CARTESIAN_POINT ( 'NONE',  ( 180.8476761818623402, 253.8486742402554910, -166.7977385971483955 ) ) ;
#31849=CARTESIAN_POINT ( 'NONE',  ( -4.232582328867905197, -278.6149089201633728, -337.4858259348673073 ) ) ;
#31850=CARTESIAN_POINT ( 'NONE',  ( -114.2697642191412655, -272.9088482181212498, -284.0992320288099791 ) ) ;
#31851=CARTESIAN_POINT ( 'NONE',  ( 31.84994229670647670, -279.9390543397678925, -298.3676068523774916 ) ) ;
#31852=CARTESIAN_POINT ( 'NONE',  ( -104.8531774944120798, -296.2762003072896846, -242.3237662583216547 ) ) ;
#31853=CARTESIAN_POINT ( 'NONE',  ( 35.42616303855504611, -293.3768198400439928, -295.5116376855012845 ) ) ;
#31854=DIRECTION ( 'NONE',  ( -1.000000000000000000, -0.000000000000000000, -0.000000000000000000 ) ) ;
#31855=CARTESIAN_POINT ( 'NONE',  ( -75.47001902956293407, -296.1291383984989238, -204.0822949002132418 ) ) ;
#31856=CARTESIAN_POINT ( 'NONE',  ( -69.12072839533406921, -287.8771842285432285, -336.9684282428895585 ) ) ;
#31857=CARTESIAN_POINT ( 'NONE',  ( 25.48506558515284937, -295.9508207140413560, -310.0009049432887878 ) ) ;
#31858=CARTESIAN_POINT ( 'NONE',  ( -1.963600746039354306, -287.8458789502048489, -205.8863748293175604 ) ) ;
#31860=CARTESIAN_POINT ( 'NONE',  ( -5.994023019284250964, -293.3954294072080984, -200.2744594085232563 ) ) ;
#31861=CARTESIAN_POINT ( 'NONE',  ( -99.66508547038839083, -285.5705881369278814, -232.1361929606052570 ) ) ;
#31862=CARTESIAN_POINT ( 'NONE',  ( -97.91052340887563332, -295.9766752593686761, -223.4419120162062882 ) ) ;
#31863=CARTESIAN_POINT ( 'NONE',  ( -86.41777221615089388, -292.1937952520814292, -211.1675960672763779 ) ) ;
#31864=CARTESIAN_POINT ( 'NONE',  ( -74.65454616443274460, -292.0615893721245016, -203.0760644864496101 ) ) ;
#31865=CARTESIAN_POINT ( 'NONE',  ( 5.846333416531644289, -288.6151341068022020, -329.2781200263282244 ) ) ;
#31868=CARTESIAN_POINT ( 'NONE',  ( 74.09727644056822271, -301.2935895614463675, -194.5614116136725045 ) ) ;
#31869=CARTESIAN_POINT ( 'NONE',  ( -68.66757489526206371, -272.4444544232246699, -200.4418753842954857 ) ) ;
#31871=CARTESIAN_POINT ( 'NONE',  ( 25.75568344301485268, -281.1211054849086963, -307.6382906422340398 ) ) ;
#31872=ORIENTED_EDGE ( 'NONE', *, *, #43435, .T. ) ;
#31873=CARTESIAN_POINT ( 'NONE',  ( -9.240139294532259129, -276.2020906246852974, -341.9839438271516201 ) ) ;
#31874=CARTESIAN_POINT ( 'NONE',  ( -92.60383411666781228, -271.6433330869302836, -221.4475517326621912 ) ) ;
#31875=CARTESIAN_POINT ( 'NONE',  ( -70.30982684041379116, -281.4733711013172410, -203.8341187175132063 ) ) ;
#31876=CARTESIAN_POINT ( 'NONE',  ( 23.46419122538822322, -274.2768113399873755, -313.0346475994430762 ) ) ;
#31877=CARTESIAN_POINT ( 'NONE',  ( -108.5639646114405963, -297.9906066198687995, -252.5749204066959237 ) ) ;
#31878=CARTESIAN_POINT ( 'NONE',  ( 9.161364539541075658, -299.7274143246822291, -197.0432256491417320 ) ) ;
#31879=CARTESIAN_POINT ( 'NONE',  ( -109.1043702041562682, -298.4791070789244714, -244.7376990471343561 ) ) ;
#31880=CARTESIAN_POINT ( 'NONE',  ( -65.58680202967329365, -271.7047737576141344, -200.4858111787266637 ) ) ;
#31881=CARTESIAN_POINT ( 'NONE',  ( 32.72439651894691082, -293.9259643279607417, -249.3388585973115141 ) ) ;
#31882=CARTESIAN_POINT ( 'NONE',  ( -57.80149485178242941, -290.3575542961208953, -199.6199712493877314 ) ) ;
#31884=CARTESIAN_POINT ( 'NONE',  ( -10.37506249526197699, -274.8869956241390469, -198.2466361817992322 ) ) ;
#31885=CARTESIAN_POINT ( 'NONE',  ( -65.81510352289728871, -273.8356662857958668, -203.1430749908509199 ) ) ;
#31886=CARTESIAN_POINT ( 'NONE',  ( 23.85053063380354743, -280.8521416932389343, -316.2828902533398718 ) ) ;
#31887=CARTESIAN_POINT ( 'NONE',  ( -34.88834522886462963, -297.0215532193161039, -345.4877409546422768 ) ) ;
#31889=CARTESIAN_POINT ( 'NONE',  ( -109.6595637643180794, -283.5992156922690128, -281.7647174284704192 ) ) ;
#31890=CARTESIAN_POINT ( 'NONE',  ( -60.68705807224014137, -281.3540195782809974, -341.8649252344125102 ) ) ;
#31891=CARTESIAN_POINT ( 'NONE',  ( 32.62767779990911521, -273.8248737225063110, -247.4009919039763190 ) ) ;
#31892=CARTESIAN_POINT ( 'NONE',  ( -43.04105364428300362, -281.9804960131575626, -195.5267823691980027 ) ) ;
#31894=CARTESIAN_POINT ( 'NONE',  ( -112.3417001281054297, -274.5519904173220311, -270.3865538441530134 ) ) ;
#31895=CARTESIAN_POINT ( 'NONE',  ( -41.13236985096396126, -272.4052040967222865, -194.2037420736955369 ) ) ;
#31897=CARTESIAN_POINT ( 'NONE',  ( -59.10917007174773374, -279.3333775728684145, -342.3069703749188761 ) ) ;
#31899=CARTESIAN_POINT ( 'NONE',  ( -96.89410921334201987, -285.8390263795151327, -316.8672979406983927 ) ) ;
#31901=CARTESIAN_POINT ( 'NONE',  ( -109.7634582419306497, -288.8031995013129176, -250.8165591967779164 ) ) ;
#31903=CARTESIAN_POINT ( 'NONE',  ( -101.8234346083377204, -294.8711233832095218, -305.4215860656804011 ) ) ;
#31904=CARTESIAN_POINT ( 'NONE',  ( 21.31917642920348754, -286.3220671818577898, -315.8763828933383593 ) ) ;
#31905=CARTESIAN_POINT ( 'NONE',  ( 79.80194596570532894, 84.98805272827966917, -300.3302785054510196 ) ) ;
#31906=CARTESIAN_POINT ( 'NONE',  ( -95.50941791035214123, -293.8995456198923648, -317.7259745329529323 ) ) ;
#31907=CARTESIAN_POINT ( 'NONE',  ( 20.94677185556329846, -286.7015515683531248, -319.6070496759664934 ) ) ;
#31908=CARTESIAN_POINT ( 'NONE',  ( 35.01907236396948520, -283.3423687231612575, -284.9285592539940808 ) ) ;
#31909=CARTESIAN_POINT ( 'NONE',  ( -27.52551098264708784, -281.1690817460281551, -345.7637356916616227 ) ) ;
#31910=CARTESIAN_POINT ( 'NONE',  ( -69.97245264539293430, -289.4943724409212109, -335.6760795783523008 ) ) ;
#31911=CARTESIAN_POINT ( 'NONE',  ( 34.22742982456013294, -283.2022142483533571, -287.5388747412744124 ) ) ;
#31912=CARTESIAN_POINT ( 'NONE',  ( -24.02609789398796636, -283.6805377689173042, -342.3006513673317386 ) ) ;
#31913=CARTESIAN_POINT ( 'NONE',  ( 20.24864189410923032, -290.2009997342684642, -318.9590532439549975 ) ) ;
#31914=CARTESIAN_POINT ( 'NONE',  ( -43.29187421240101230, -298.1457895272055794, -193.5381517441040842 ) ) ;
#31915=CARTESIAN_POINT ( 'NONE',  ( -35.52378678070758156, -274.0743408453358825, -193.3694505866060922 ) ) ;
#31916=CARTESIAN_POINT ( 'NONE',  ( -49.99173294697245495, -293.8699949332213350, -196.7435368656326489 ) ) ;
#31918=CARTESIAN_POINT ( 'NONE',  ( -85.33152481854864391, -281.9090924074130839, -210.2361428286349110 ) ) ;
#31919=CARTESIAN_POINT ( 'NONE',  ( -31.61595600124092442, -274.9799995323535882, -345.3607659508787719 ) ) ;
#31921=CARTESIAN_POINT ( 'NONE',  ( -110.8448982739032687, -295.2085583523438004, -250.0735484861346549 ) ) ;
#31922=CARTESIAN_POINT ( 'NONE',  ( -108.4916734135219656, -291.8939093006709982, -290.1482683914920813 ) ) ;
#31923=CARTESIAN_POINT ( 'NONE',  ( -51.57319391114928209, -273.2140119269045044, -198.6059989695407921 ) ) ;
#31924=CARTESIAN_POINT ( 'NONE',  ( -110.6646592534776232, -292.1687075913327476, -262.9819976625192339 ) ) ;
#31925=CARTESIAN_POINT ( 'NONE',  ( -25.38243844869774435, -293.1494479978140362, -198.0572463151052602 ) ) ;
#31926=CARTESIAN_POINT ( 'NONE',  ( -78.92774084220380360, -285.3815113308673403, -331.5867272440648321 ) ) ;
#31928=CARTESIAN_POINT ( 'NONE',  ( -47.68176297217866022, -293.3485544582074454, -194.5998119806215527 ) ) ;
#31929=CARTESIAN_POINT ( 'NONE',  ( -90.45570503368409732, -292.6344998693948583, -215.2221533620264324 ) ) ;
#31930=CARTESIAN_POINT ( 'NONE',  ( -3.145635356501999880, -294.4203921897134819, -334.8563050794364244 ) ) ;
#31931=CARTESIAN_POINT ( 'NONE',  ( 32.83726428960925148, -289.2069678626473888, -243.7587688623997906 ) ) ;
#31932=CARTESIAN_POINT ( 'NONE',  ( 38.66818699411951599, -281.8737954578546692, -282.7519086214052777 ) ) ;
#31933=CARTESIAN_POINT ( 'NONE',  ( -4.174018851904285121, -296.5441181210520654, -194.8118598026143218 ) ) ;
#31934=CARTESIAN_POINT ( 'NONE',  ( -109.3037131088121612, -284.0370359753096636, -297.9043881315205340 ) ) ;
#31935=CARTESIAN_POINT ( 'NONE',  ( -9.348653367303350947, -278.6643636632716152, -339.5720734106865280 ) ) ;
#31936=EDGE_CURVE ( 'NONE', #69774, #78913, #15765, .T. ) ;
#31937=CARTESIAN_POINT ( 'NONE',  ( -45.69984345545591253, -281.9552266982748847, -343.3320169154444557 ) ) ;
#31938=CARTESIAN_POINT ( 'NONE',  ( 6.398740975593778302, -284.6456943985136263, -209.3728041133678346 ) ) ;
#31939=CARTESIAN_POINT ( 'NONE',  ( -39.94463377582687258, -275.2240852786313212, -346.0940523342308097 ) ) ;
#31940=DIRECTION ( 'NONE',  ( -1.000000000000000000, -0.000000000000000000, -0.000000000000000000 ) ) ;
#31941=CARTESIAN_POINT ( 'NONE',  ( -51.03557406219254489, -282.7394153745999574, -342.1794875296856731 ) ) ;
#31942=CARTESIAN_POINT ( 'NONE',  ( -45.24773267194631643, -281.1593317729493720, -194.1145467414838208 ) ) ;
#31943=CARTESIAN_POINT ( 'NONE',  ( 30.15008815713381907, -287.0867521836036644, -307.0465474153882610 ) ) ;
#31944=CARTESIAN_POINT ( 'NONE',  ( -39.69916556040571010, -296.8422720438277906, -344.3495036058563983 ) ) ;
#31945=CARTESIAN_POINT ( 'NONE',  ( 19.29637331677102452, -277.8516235887336165, -321.3568127997767192 ) ) ;
#31946=CARTESIAN_POINT ( 'NONE',  ( 28.07215220619743334, -276.3448830913356460, -230.5820953063862646 ) ) ;
#31947=CARTESIAN_POINT ( 'NONE',  ( -96.88692640626264563, -277.7955435774362627, -312.6127471272376965 ) ) ;
#31948=CARTESIAN_POINT ( 'NONE',  ( -67.58300229782625479, -299.6546725945485150, -201.8964377673428601 ) ) ;
#31949=CARTESIAN_POINT ( 'NONE',  ( 27.97982403285748276, -285.0635795132146200, -233.7430230635522150 ) ) ;
#31950=CARTESIAN_POINT ( 'NONE',  ( -112.8759555970320463, -292.2841868556409395, -259.9233491448626978 ) ) ;
#31951=CARTESIAN_POINT ( 'NONE',  ( -36.18752924115639757, -290.9872492672425892, -197.0485618474658907 ) ) ;
#31953=CARTESIAN_POINT ( 'NONE',  ( -30.80085406721504171, -291.8038276289709074, -197.6335109850780611 ) ) ;
#31955=CARTESIAN_POINT ( 'NONE',  ( -45.97725273223464626, -290.2387521758650450, -346.6171789037773010 ) ) ;
#31956=CARTESIAN_POINT ( 'NONE',  ( -54.52478548652082679, -280.4770368167814922, -199.2551044200497188 ) ) ;
#31957=CARTESIAN_POINT ( 'NONE',  ( -105.6884919800661322, -295.0213861220104263, -305.2661931755152409 ) ) ;
#31958=CARTESIAN_POINT ( 'NONE',  ( 32.61584204828126587, -287.7934497353121515, -238.3071889476116212 ) ) ;
#31959=CARTESIAN_POINT ( 'NONE',  ( 5.164463920278626219, -286.9429476111998270, -206.1184260131755934 ) ) ;
#31960=CARTESIAN_POINT ( 'NONE',  ( -88.90621632563291143, -284.1342473866651517, -322.1349688073923971 ) ) ;
#31961=CARTESIAN_POINT ( 'NONE',  ( -95.69098327614956645, -240.0217764934971001, -341.7741963911435619 ) ) ;
#31962=CARTESIAN_POINT ( 'NONE',  ( -112.8381603000581350, -269.0091090816746942, -295.8145170300798554 ) ) ;
#31963=CARTESIAN_POINT ( 'NONE',  ( -89.05334355809267777, -229.2207001999348677, -344.3638864873447005 ) ) ;
#31965=CARTESIAN_POINT ( 'NONE',  ( -69.33123261485080491, -276.6812832171280547, -336.1721864582053740 ) ) ;
#31966=CARTESIAN_POINT ( 'NONE',  ( -61.90630208261759293, -276.2992970384053706, -339.4861145567745666 ) ) ;
#31967=CARTESIAN_POINT ( 'NONE',  ( -99.54745726220131985, -272.8218831187957107, -224.9275258499349945 ) ) ;
#31968=CARTESIAN_POINT ( 'NONE',  ( -109.1411030854801680, -269.7224105353499226, -295.4917919841202547 ) ) ;
#31969=CARTESIAN_POINT ( 'NONE',  ( -111.6998803920500194, -277.0096726131649802, -288.4204631147621853 ) ) ;
#31970=EDGE_LOOP ( 'NONE', ( #61434, #14826, #51298, #60157 ) ) ;
#31971=CARTESIAN_POINT ( 'NONE',  ( -108.1696792713219537, -291.2815145907476335, -252.3829820995457283 ) ) ;
#31972=CARTESIAN_POINT ( 'NONE',  ( -34.77642259965058713, -298.8863312046613601, -193.5222535600145477 ) ) ;
#31973=CARTESIAN_POINT ( 'NONE',  ( -73.25748586429388354, -298.0816139074282205, -202.2612753892758235 ) ) ;
#31974=CARTESIAN_POINT ( 'NONE',  ( -35.64848614041083152, -295.1970355033479336, -343.3539746444233742 ) ) ;
#31976=CARTESIAN_POINT ( 'NONE',  ( -81.68114528108452532, -279.5708025579765490, -331.5438590043891054 ) ) ;
#31977=CARTESIAN_POINT ( 'NONE',  ( 9.166618469806152802, -281.9401319130670345, -331.6514369918072020 ) ) ;
#31978=CARTESIAN_POINT ( 'NONE',  ( -83.18941239012731614, -278.7765105923450051, -327.6297055266257985 ) ) ;
#31979=CARTESIAN_POINT ( 'NONE',  ( 22.73089993036286671, -277.9420915592434653, -316.9145473372589095 ) ) ;
#31980=CARTESIAN_POINT ( 'NONE',  ( -34.43264168466875930, -296.6639937130342446, -196.7726070210977127 ) ) ;
#31982=CARTESIAN_POINT ( 'NONE',  ( -97.64763201024906891, -278.1465152655208044, -311.4974107704672406 ) ) ;
#31983=CARTESIAN_POINT ( 'NONE',  ( 17.96624922607475483, -275.6223732806200246, -216.9444315659675055 ) ) ;
#31984=CARTESIAN_POINT ( 'NONE',  ( -5.844916577696278814, -287.3314721402164764, -340.0837893332466138 ) ) ;
#31985=CARTESIAN_POINT ( 'NONE',  ( -38.35657888232754686, -276.0395859197232085, -195.3679804698540181 ) ) ;
#31986=CARTESIAN_POINT ( 'NONE',  ( 23.04116999833489388, -274.7571934940123697, -317.2066346513356052 ) ) ;
#31988=CARTESIAN_POINT ( 'NONE',  ( -70.05382376342366513, -288.6916700083741603, -335.8159647033965030 ) ) ;
#31989=CARTESIAN_POINT ( 'NONE',  ( -110.8261557548513139, -284.1876919767618688, -247.5247831497662219 ) ) ;
#31990=CARTESIAN_POINT ( 'NONE',  ( 23.40381856939280070, -280.3733317625773225, -312.6453463948412264 ) ) ;
#31991=CARTESIAN_POINT ( 'NONE',  ( -5.285548949164077470, -279.0572488752454205, -204.1208123464883784 ) ) ;
#31992=CARTESIAN_POINT ( 'NONE',  ( -41.37701451950836429, -284.0808237527692768, -196.0178244446223630 ) ) ;
#31993=CARTESIAN_POINT ( 'NONE',  ( -62.47099950814151725, -291.3791134923286563, -341.0802947170757307 ) ) ;
#31994=CARTESIAN_POINT ( 'NONE',  ( -109.6747952858519994, -279.5928836896200664, -282.8873786463282158 ) ) ;
#31995=CARTESIAN_POINT ( 'NONE',  ( 138.5464851867201617, 180.7133913485274093, -241.3450705794696205 ) ) ;
#31996=CARTESIAN_POINT ( 'NONE',  ( -24.68671676498891543, -281.2932795958516863, -345.5564807554345066 ) ) ;
#31997=CARTESIAN_POINT ( 'NONE',  ( 33.55350136275063022, -295.2337867552957960, -245.7322287256875484 ) ) ;
#31998=CARTESIAN_POINT ( 'NONE',  ( -74.49267372065884274, -277.8048166309754947, -204.0755299897761006 ) ) ;
#31999=CARTESIAN_POINT ( 'NONE',  ( -65.85659864257682727, -285.4244470034578853, -339.9229974522152133 ) ) ;
#32001=CARTESIAN_POINT ( 'NONE',  ( -76.44537179901922741, -293.4540489764297604, -205.6461673090609850 ) ) ;
#32002=CARTESIAN_POINT ( 'NONE',  ( 21.57826782591973114, -274.1893918477034617, -316.7869431542051188 ) ) ;
#32003=CARTESIAN_POINT ( 'NONE',  ( 2.665679482944644629, -285.7715786691190942, -204.7595296100580526 ) ) ;
#32004=CARTESIAN_POINT ( 'NONE',  ( -90.37722399140584173, -289.6856194578234636, -219.0417880621873792 ) ) ;
#32006=CARTESIAN_POINT ( 'NONE',  ( 20.39958492059878026, -274.8742674453797008, -315.8477130392956269 ) ) ;
#32007=CARTESIAN_POINT ( 'NONE',  ( -47.99330059431824225, -293.3285065996022354, -343.8803275178525496 ) ) ;
#32010=CARTESIAN_POINT ( 'NONE',  ( 25.92896271279305154, -291.4638424328961719, -227.6121752193068914 ) ) ;
#32011=CARTESIAN_POINT ( 'NONE',  ( -105.3425452505865962, -286.5345412973486532, -241.5534608477831853 ) ) ;
#32012=CARTESIAN_POINT ( 'NONE',  ( -2.288377031563566533, -286.8345532044896800, -337.7795023884337979 ) ) ;
#32013=CARTESIAN_POINT ( 'NONE',  ( 0.4558526818627712252, -287.9913483902537337, -207.1612409286476009 ) ) ;
#32015=CARTESIAN_POINT ( 'NONE',  ( 35.79188056954839681, -288.3996901881048984, -273.7571519457596310 ) ) ;
#32016=CARTESIAN_POINT ( 'NONE',  ( 29.42954581387986224, -295.0702523157631276, -235.3202499388733884 ) ) ;
#32018=CARTESIAN_POINT ( 'NONE',  ( 13.96946583782010620, -287.9580253817053404, -213.4113852361003012 ) ) ;
#32019=CARTESIAN_POINT ( 'NONE',  ( -103.7224080617017847, -276.1560174391986493, -306.4570430947074442 ) ) ;
#32021=CARTESIAN_POINT ( 'NONE',  ( -95.19209669629114501, -278.1979918697487051, -321.1457210475748525 ) ) ;
#32023=CARTESIAN_POINT ( 'NONE',  ( 22.86143368094143113, -280.5762170911689850, -222.3680122932001666 ) ) ;
#32024=CARTESIAN_POINT ( 'NONE',  ( -66.23208441319731321, -299.6519751437826358, -201.5338523080350228 ) ) ;
#32026=CARTESIAN_POINT ( 'NONE',  ( -19.31102908077654945, -284.2839792367648215, -197.5607364776439852 ) ) ;
#32028=CARTESIAN_POINT ( 'NONE',  ( -109.3763362795433380, -276.4583063858643754, -288.3545119142069666 ) ) ;
#32029=CARTESIAN_POINT ( 'NONE',  ( 16.37555915972660259, -280.2894872585930557, -322.7751182829704817 ) ) ;
#32031=CARTESIAN_POINT ( 'NONE',  ( -14.81303407438512920, -275.2454511245171034, -343.3216278436320295 ) ) ;
#32033=CARTESIAN_POINT ( 'NONE',  ( -78.31935103185020353, -297.1342574607348865, -331.6725587702009648 ) ) ;
#32034=CARTESIAN_POINT ( 'NONE',  ( 6.736064839718973296, -281.3887484030951782, -333.1846588522895445 ) ) ;
#32035=CARTESIAN_POINT ( 'NONE',  ( -57.98253738569656690, -298.7201153642972713, -200.0947370821152731 ) ) ;
#32036=CARTESIAN_POINT ( 'NONE',  ( -96.97257719552548849, -298.5138026828739726, -222.4293250339174790 ) ) ;
#32037=CARTESIAN_POINT ( 'NONE',  ( -29.98351685608239592, -273.8145655281006725, -197.7116539398417672 ) ) ;
#32038=CARTESIAN_POINT ( 'NONE',  ( 37.42006093121500498, -295.6290118130862083, -276.3343691895940424 ) ) ;
#32039=CARTESIAN_POINT ( 'NONE',  ( 30.13053733563801018, -287.2370886836560544, -233.1493159620859501 ) ) ;
#32040=CARTESIAN_POINT ( 'NONE',  ( -110.6821945957990749, -276.8643752507669547, -252.1288293495414052 ) ) ;
#32041=CARTESIAN_POINT ( 'NONE',  ( -106.0031489579009474, -290.8354881621830259, -235.3923703725757832 ) ) ;
#32043=CARTESIAN_POINT ( 'NONE',  ( 17.07345212859976513, -285.9111754903252063, -221.3281124510065752 ) ) ;
#32044=CARTESIAN_POINT ( 'NONE',  ( 37.24020743009980805, -291.4443189532779570, -261.9755118474089954 ) ) ;
#32045=EDGE_LOOP ( 'NONE', ( #46274, #43050 ) ) ;
#32046=CARTESIAN_POINT ( 'NONE',  ( 207.9738562182569979, 296.4636489450776367, -53.99999999999996447 ) ) ;
#32047=CARTESIAN_POINT ( 'NONE',  ( -10.70750508443766336, -288.2029641790746837, -338.4492520772749913 ) ) ;
#32049=CARTESIAN_POINT ( 'NONE',  ( -74.15258365676309893, -284.4699494192838642, -337.7834632798797543 ) ) ;
#32050=CARTESIAN_POINT ( 'NONE',  ( -25.04727851266873273, -291.2640311931895667, -194.5873269362672318 ) ) ;
#32051=CARTESIAN_POINT ( 'NONE',  ( 22.23692858310425535, -282.5093135698551805, -222.8343035938656271 ) ) ;
#32052=CARTESIAN_POINT ( 'NONE',  ( -35.36565949769887851, -281.3916044359212947, -193.8667371012928413 ) ) ;
#32053=CARTESIAN_POINT ( 'NONE',  ( -76.12892137985416241, -283.4192246183785642, -332.2638588864539315 ) ) ;
#32054=CARTESIAN_POINT ( 'NONE',  ( -100.7506633848914532, -297.1291343217696976, -226.6538149999235259 ) ) ;
#32055=CARTESIAN_POINT ( 'NONE',  ( -105.8821865621944482, -274.2210059718004800, -243.6981114570576210 ) ) ;
#32056=CARTESIAN_POINT ( 'NONE',  ( 22.32338184616281396, -290.9563049268516011, -225.5066332715741169 ) ) ;
#32057=CARTESIAN_POINT ( 'NONE',  ( -40.77825468412755328, -272.8030252614012738, -196.9945683960216627 ) ) ;
#32060=CARTESIAN_POINT ( 'NONE',  ( -72.05922115847914711, -285.4351851772863142, -336.2094887573258575 ) ) ;
#32061=CARTESIAN_POINT ( 'NONE',  ( -53.21179875707857576, -296.3305898399432863, -345.4463168423347383 ) ) ;
#32062=CARTESIAN_POINT ( 'NONE',  ( -108.8179802862372156, -285.0008273800320353, -285.7513601206922544 ) ) ;
#32063=CARTESIAN_POINT ( 'NONE',  ( 10.37040957557863230, -275.4709780767523171, -330.5652885095761917 ) ) ;
#32064=CARTESIAN_POINT ( 'NONE',  ( -2.109941594086266914, -293.1575623248617717, -201.9940674419532058 ) ) ;
#32065=CARTESIAN_POINT ( 'NONE',  ( 35.58887856450918008, -285.9537473155775160, -290.9375527471842133 ) ) ;
#32066=CARTESIAN_POINT ( 'NONE',  ( -3.334518190640860524, -292.8221923266876843, -201.2867855567963602 ) ) ;
#32067=CARTESIAN_POINT ( 'NONE',  ( -95.78269330669334636, -290.2708205165193363, -314.1625476471908769 ) ) ;
#32070=CARTESIAN_POINT ( 'NONE',  ( -21.32748300042747047, -109.1711728762462599, -358.9589870467152082 ) ) ;
#32071=CARTESIAN_POINT ( 'NONE',  ( -95.30271994553761772, -286.7486808275992871, -220.6509291276668705 ) ) ;
#32072=CARTESIAN_POINT ( 'NONE',  ( -111.2869819898779866, -275.6237833571633473, -305.9350535429201159 ) ) ;
#32074=CARTESIAN_POINT ( 'NONE',  ( -61.65013534321383304, -282.2957530560925079, -339.5761776175779119 ) ) ;
#32075=CARTESIAN_POINT ( 'NONE',  ( -113.0456101871530592, -278.0434275631234868, -284.3857043565927256 ) ) ;
#32076=CARTESIAN_POINT ( 'NONE',  ( -39.78600746564308821, -282.0215683001354705, -195.5548766155741021 ) ) ;
#32077=CARTESIAN_POINT ( 'NONE',  ( -75.54299273995306407, -209.4449673374598149, -355.7036186976513932 ) ) ;
#32078=CARTESIAN_POINT ( 'NONE',  ( -37.33268361118738454, -281.6267396580638547, -346.7848558294755890 ) ) ;
#32079=CARTESIAN_POINT ( 'NONE',  ( 20.81214822973163336, -284.9250317276720352, -223.5436714221757484 ) ) ;
#32080=CARTESIAN_POINT ( 'NONE',  ( -108.0229871219324025, -274.7654568338024887, -242.9317705756486419 ) ) ;
#32081=CARTESIAN_POINT ( 'NONE',  ( -45.09103359206184081, -295.6451422462782261, -343.0610436786520268 ) ) ;
#32083=CARTESIAN_POINT ( 'NONE',  ( -3.393670155583646597, -291.1950900457537728, -205.1784919218372067 ) ) ;
#32084=CARTESIAN_POINT ( 'NONE',  ( -97.84356587086362822, -278.5682003954476045, -317.8251783733547882 ) ) ;
#32085=CARTESIAN_POINT ( 'NONE',  ( 19.85550291320718941, -274.9116816451208933, -224.9816635841000618 ) ) ;
#32086=CARTESIAN_POINT ( 'NONE',  ( 21.48464173678410916, -275.1373264880589886, -319.5643090745783752 ) ) ;
#32088=CARTESIAN_POINT ( 'NONE',  ( -25.24924945877150861, -272.2060155210314747, -196.2903500954780327 ) ) ;
#32089=CARTESIAN_POINT ( 'NONE',  ( 24.42080315769786125, -295.5793515982531403, -315.3720463854793934 ) ) ;
#32094=CARTESIAN_POINT ( 'NONE',  ( -80.79836427686932154, -284.7369270057944277, -329.4644607051857861 ) ) ;
#32095=CARTESIAN_POINT ( 'NONE',  ( 17.11590623432395475, -284.0491827155746591, -323.4301284291572074 ) ) ;
#32096=CARTESIAN_POINT ( 'NONE',  ( -109.0272987253608363, -284.0893804607008519, -256.0409356430674848 ) ) ;
#32097=CARTESIAN_POINT ( 'NONE',  ( 14.27647268826083859, -274.7122533925004859, -323.1769808572024658 ) ) ;
#32098=CARTESIAN_POINT ( 'NONE',  ( -56.61717963045364144, -285.1637002456756704, -342.0501782889522815 ) ) ;
#32099=CARTESIAN_POINT ( 'NONE',  ( -98.23252094285805924, -276.4599854975878657, -311.8703421778951110 ) ) ;
#32102=CARTESIAN_POINT ( 'NONE',  ( 35.32510718580935816, -276.5046316906208972, -260.6780818678755622 ) ) ;
#32106=CARTESIAN_POINT ( 'NONE',  ( -36.76405678750610662, -280.8620680775485425, -193.5117469678797022 ) ) ;
#32107=CARTESIAN_POINT ( 'NONE',  ( -64.72629259894902987, -280.1964588649249777, -198.4049243463213088 ) ) ;
#32110=CARTESIAN_POINT ( 'NONE',  ( 82.64890176555634582, -299.5541904835127980, -195.3611179825600175 ) ) ;
#32111=CARTESIAN_POINT ( 'NONE',  ( -24.02664636421022237, -288.0807479783902636, -195.7221530634781459 ) ) ;
#32112=CARTESIAN_POINT ( 'NONE',  ( -26.19286370360628169, -294.1037444226016646, -342.6681382016752764 ) ) ;
#32113=CARTESIAN_POINT ( 'NONE',  ( -112.7696401988369814, -289.7125050854687629, -285.3924768128118217 ) ) ;
#32115=CARTESIAN_POINT ( 'NONE',  ( 33.24670168618867905, -285.5005518376915461, -248.0643989013786097 ) ) ;
#32116=CARTESIAN_POINT ( 'NONE',  ( 35.58255743526108006, -285.9928287594933067, -260.1177032164763432 ) ) ;
#32117=CARTESIAN_POINT ( 'NONE',  ( -73.09709437192304904, -289.8116019873651794, -205.4997853387870066 ) ) ;
#32118=CARTESIAN_POINT ( 'NONE',  ( -25.09056769541773235, -287.4167986635021634, -197.9421444574102509 ) ) ;
#32119=CARTESIAN_POINT ( 'NONE',  ( -112.2127695572321500, -276.6084302456295632, -265.9652553019528796 ) ) ;
#32120=CARTESIAN_POINT ( 'NONE',  ( 36.00873599911082579, -286.2139928166764662, -291.0524191956897084 ) ) ;
#32121=CARTESIAN_POINT ( 'NONE',  ( 33.94000919001867800, -289.2491378173115208, -246.8731416063353947 ) ) ;
#32122=CARTESIAN_POINT ( 'NONE',  ( 24.85504240161681366, -284.9816810451083029, -228.1291856884065226 ) ) ;
#32123=CARTESIAN_POINT ( 'NONE',  ( 35.66462184815443948, -282.5775475765608462, -276.7598081705659183 ) ) ;
#32124=CARTESIAN_POINT ( 'NONE',  ( 20.10476282909932166, -290.2212647467921443, -318.8372185212502927 ) ) ;
#32127=CARTESIAN_POINT ( 'NONE',  ( -62.39115482748979957, -299.6489439279044973, -199.0740994153643442 ) ) ;
#32128=CARTESIAN_POINT ( 'NONE',  ( 29.57710527583184756, -279.1031206910064384, -236.3803571566485857 ) ) ;
#32129=CARTESIAN_POINT ( 'NONE',  ( -50.52857049235809228, -291.0850188997316650, -194.6626023429500094 ) ) ;
#32130=CARTESIAN_POINT ( 'NONE',  ( -110.6011763037998747, -294.8303284794328647, -279.6869412284991085 ) ) ;
#32131=CARTESIAN_POINT ( 'NONE',  ( 34.41833540617255238, -280.4448749674814394, -286.2274590782195673 ) ) ;
#32132=CARTESIAN_POINT ( 'NONE',  ( -68.87066569254632498, -271.7142674303379408, -202.9139362639011495 ) ) ;
#32133=CARTESIAN_POINT ( 'NONE',  ( -63.73052980004775492, -296.7185716184507100, -339.0071099239967225 ) ) ;
#32135=CARTESIAN_POINT ( 'NONE',  ( 97.67869099132846600, -298.1933505581249619, -194.0885504402530728 ) ) ;
#32136=CARTESIAN_POINT ( 'NONE',  ( 24.87193957083375295, -292.3769067849592034, -314.0122142888834560 ) ) ;
#32137=CARTESIAN_POINT ( 'NONE',  ( -60.46116585165769663, -293.1717801410790685, -200.4444552939437187 ) ) ;
#32139=CARTESIAN_POINT ( 'NONE',  ( 30.00038310982760947, -293.9703699323951014, -241.6370488712062752 ) ) ;
#32140=DIRECTION ( 'NONE',  ( -0.000000000000000000, 0.000000000000000000, 1.000000000000000000 ) ) ;
#32141=CARTESIAN_POINT ( 'NONE',  ( -106.7228214564766517, -282.1882831759584178, -299.8999288511420218 ) ) ;
#32142=CARTESIAN_POINT ( 'NONE',  ( -26.20740738324616714, -294.9064477241673217, -342.5069946843668731 ) ) ;
#32143=CARTESIAN_POINT ( 'NONE',  ( 33.56592810279381212, -281.9357346024767708, -300.5157485781939499 ) ) ;
#32144=CARTESIAN_POINT ( 'NONE',  ( 9.903215597816359406, -282.6168194147061854, -211.3260124695724471 ) ) ;
#32145=CARTESIAN_POINT ( 'NONE',  ( -26.61985071651751156, -285.8515771332424151, -194.0791202020755861 ) ) ;
#32146=CARTESIAN_POINT ( 'NONE',  ( -93.92647831743205700, -289.2327514552350181, -221.3897865101162097 ) ) ;
#32147=CARTESIAN_POINT ( 'NONE',  ( -34.52412969220306138, -281.4972230269272586, -346.6157509629684910 ) ) ;
#32148=CARTESIAN_POINT ( 'NONE',  ( -40.34049286915740140, -288.0093238300307235, -347.0063840666759347 ) ) ;
#32150=CARTESIAN_POINT ( 'NONE',  ( -70.06062047065620391, -297.0907504691072631, -336.5117995295676110 ) ) ;
#32151=CARTESIAN_POINT ( 'NONE',  ( -71.29260842501039974, -278.9169105144516152, -338.8150595858230076 ) ) ;
#32152=CARTESIAN_POINT ( 'NONE',  ( 37.96226306148032137, -291.6077645447603572, -273.1395938017559502 ) ) ;
#32153=CARTESIAN_POINT ( 'NONE',  ( -22.18587604685646397, -279.9182442886329341, -198.8782400538389368 ) ) ;
#32154=CARTESIAN_POINT ( 'NONE',  ( 36.70357884842792373, -293.4534699618284321, -249.1873445060794268 ) ) ;
#32155=CARTESIAN_POINT ( 'NONE',  ( -110.3238210573160814, -282.8839533935214945, -250.5962620008469059 ) ) ;
#32156=CARTESIAN_POINT ( 'NONE',  ( -28.80276998113174969, -278.9441809999948418, -344.9256331223715506 ) ) ;
#32157=CARTESIAN_POINT ( 'NONE',  ( 35.77039601752356646, -292.5445027382672265, -265.3120231461800813 ) ) ;
#32159=CARTESIAN_POINT ( 'NONE',  ( -101.1489920581274617, -271.0844958157555311, -230.6287895603641687 ) ) ;
#32163=CARTESIAN_POINT ( 'NONE',  ( 32.40368120952480524, -293.3479379400545781, -292.1227866632826817 ) ) ;
#32165=CARTESIAN_POINT ( 'NONE',  ( -92.08974858914540107, -293.4094976428775681, -313.9805196606274080 ) ) ;
#32166=CARTESIAN_POINT ( 'NONE',  ( -101.0688888548078666, -272.3171808282273219, -227.3361863632982534 ) ) ;
#32167=CARTESIAN_POINT ( 'NONE',  ( 34.38603150638219574, -288.5286359645543826, -243.7447548483897322 ) ) ;
#32168=CARTESIAN_POINT ( 'NONE',  ( 31.39868659444720222, -287.7126360876585522, -294.9326307103727345 ) ) ;
#32170=CARTESIAN_POINT ( 'NONE',  ( -97.44001153033948981, -279.4820731503508000, -313.0315984227354988 ) ) ;
#32171=CARTESIAN_POINT ( 'NONE',  ( -36.49091421304517269, -299.8230862102235506, -196.3475185273377122 ) ) ;
#32172=CARTESIAN_POINT ( 'NONE',  ( -96.71793929998518990, -277.9476640710905144, -227.2149393871871723 ) ) ;
#32174=CARTESIAN_POINT ( 'NONE',  ( -114.1808714800626916, -272.4572214948289002, -264.6241286613252441 ) ) ;
#32175=CARTESIAN_POINT ( 'NONE',  ( -60.73423236463455765, -293.6665821841398838, -199.6380524494565520 ) ) ;
#32176=CARTESIAN_POINT ( 'NONE',  ( 22.46734290608615581, -294.5138773816356093, -223.1246125363533395 ) ) ;
#32178=CARTESIAN_POINT ( 'NONE',  ( -107.0467789165242891, -290.9100151247752706, -292.5533464571436753 ) ) ;
#32180=CARTESIAN_POINT ( 'NONE',  ( -27.97787172230660246, -290.3092628590002278, -195.1243673037924680 ) ) ;
#32181=CARTESIAN_POINT ( 'NONE',  ( -77.52006940727925155, -297.1636004414818899, -209.3267083803866910 ) ) ;
#32183=CARTESIAN_POINT ( 'NONE',  ( -108.1478418983590757, -291.7079662112038250, -298.8075244133791557 ) ) ;
#32184=CARTESIAN_POINT ( 'NONE',  ( -2.602324593224680793, -297.1233781216987495, -342.4248175857292154 ) ) ;
#32185=CARTESIAN_POINT ( 'NONE',  ( -38.68267965962606780, -288.0354893360201345, -195.5270013178786428 ) ) ;
#32186=CARTESIAN_POINT ( 'NONE',  ( 28.25556057384566344, -273.0708667715167053, -234.2387795365413865 ) ) ;
#32187=CARTESIAN_POINT ( 'NONE',  ( -3.470884329266651580, -276.4229604262348516, -204.0589377984777286 ) ) ;
#32188=CARTESIAN_POINT ( 'NONE',  ( -22.42870598061681520, -290.3244204270775413, -197.4302136928437790 ) ) ;
#32189=CARTESIAN_POINT ( 'NONE',  ( -112.8459830926621663, -280.3250994698489649, -277.2428428359876875 ) ) ;
#32192=CARTESIAN_POINT ( 'NONE',  ( 9.968359227623851737, -281.7288842460441174, -326.1560474453642655 ) ) ;
#32193=CARTESIAN_POINT ( 'NONE',  ( -91.10250224597039903, -278.8736926504901135, -325.1279636279851957 ) ) ;
#32194=CARTESIAN_POINT ( 'NONE',  ( 37.75324310583263809, -280.5372181615706495, -285.4858732045136662 ) ) ;
#32195=CARTESIAN_POINT ( 'NONE',  ( 63.42269039470908609, 47.43533074464846777, -315.9655852024159230 ) ) ;
#32196=CARTESIAN_POINT ( 'NONE',  ( 32.80961911128900255, -276.8924477317431752, -301.5318193105213140 ) ) ;
#32197=CARTESIAN_POINT ( 'NONE',  ( -15.99008950958257991, -275.8433804732711110, -197.0477229558706256 ) ) ;
#32198=CARTESIAN_POINT ( 'NONE',  ( -54.42813229853333468, -297.7662352645559167, -345.3683826091709648 ) ) ;
#32202=CARTESIAN_POINT ( 'NONE',  ( -99.09477969312752066, -291.0876510141624181, -309.8678672499180493 ) ) ;
#32203=CARTESIAN_POINT ( 'NONE',  ( -40.27687523391615798, -290.8486774883558610, -346.3039873528174439 ) ) ;
#32204=CARTESIAN_POINT ( 'NONE',  ( -110.0734738020615140, -289.9975223248215457, -263.0138895065859401 ) ) ;
#32205=CARTESIAN_POINT ( 'NONE',  ( -80.89819907993499726, -284.9861552802685765, -206.8747494338723527 ) ) ;
#32207=CARTESIAN_POINT ( 'NONE',  ( -2.063978847144392947, -280.9767570088134221, -335.1978020052873717 ) ) ;
#32208=CARTESIAN_POINT ( 'NONE',  ( 36.50067403360087326, -289.3136365659321996, -262.7342406910485693 ) ) ;
#32209=CARTESIAN_POINT ( 'NONE',  ( -21.25554649829815546, -281.3220712254017712, -342.3298469887318447 ) ) ;
#32211=CARTESIAN_POINT ( 'NONE',  ( 32.43959880854713163, -282.5613434196513367, -247.1397469063622623 ) ) ;
#32212=CARTESIAN_POINT ( 'NONE',  ( 37.88013025497256336, -288.6855003090064429, -285.6743948231272725 ) ) ;
#32213=CARTESIAN_POINT ( 'NONE',  ( -94.84317303782539454, -279.6796644029840877, -225.2680486695198852 ) ) ;
#32214=CARTESIAN_POINT ( 'NONE',  ( -96.26356086346071095, -290.0089469606664920, -221.3896212359633182 ) ) ;
#32215=CARTESIAN_POINT ( 'NONE',  ( -111.7160819607365738, -285.1122859357790276, -289.7163666339131964 ) ) ;
#32216=CARTESIAN_POINT ( 'NONE',  ( -2.256567359835757181, -286.9962189965971220, -201.8733146190533034 ) ) ;
#32217=CARTESIAN_POINT ( 'NONE',  ( -86.92728023471225640, -283.9318838215097003, -324.0051758269629545 ) ) ;
#32220=CARTESIAN_POINT ( 'NONE',  ( -25.24241823611405877, -294.0652479960531309, -195.5686527472780085 ) ) ;
#32221=CARTESIAN_POINT ( 'NONE',  ( 34.99188720886146342, -291.9189866085632161, -245.2777599125674044 ) ) ;
#32222=CARTESIAN_POINT ( 'NONE',  ( 32.31830253633833649, -274.9098179559817368, -292.9640486980184164 ) ) ;
#32223=CARTESIAN_POINT ( 'NONE',  ( -32.02784585440693377, -294.3353892984665663, -347.0886022834904452 ) ) ;
#32224=CARTESIAN_POINT ( 'NONE',  ( -109.3843267870809228, -289.2347090133541769, -254.8508730272920388 ) ) ;
#32225=CARTESIAN_POINT ( 'NONE',  ( 19.59851942928052537, -292.4535114628120027, -317.6452105804276016 ) ) ;
#32227=CARTESIAN_POINT ( 'NONE',  ( -44.35333418936818362, -293.1667142387942704, -197.2486277647709016 ) ) ;
#32230=CARTESIAN_POINT ( 'NONE',  ( 36.79377204633100007, -291.7119545663063036, -282.8470202735847465 ) ) ;
#32231=CARTESIAN_POINT ( 'NONE',  ( 36.17919655412337221, -295.7434367353993707, -285.2464710003911819 ) ) ;
#32232=CARTESIAN_POINT ( 'NONE',  ( 35.35923419026552494, -288.6095270909180499, -279.1918935565688002 ) ) ;
#32233=CARTESIAN_POINT ( 'NONE',  ( -70.81702276271015251, -279.4714406329405278, -337.8726694500839471 ) ) ;
#32234=CARTESIAN_POINT ( 'NONE',  ( -14.72166629277199945, -275.5604466277056872, -343.6036917696333148 ) ) ;
#32235=CARTESIAN_POINT ( 'NONE',  ( -34.04527844338633003, -297.2896107109601189, -193.5230290258803620 ) ) ;
#32236=CARTESIAN_POINT ( 'NONE',  ( -65.33540394513283900, -277.7632060720709433, -201.3852762297734387 ) ) ;
#32237=CARTESIAN_POINT ( 'NONE',  ( -92.76626186915059691, -276.2298706324993418, -322.7298619205337218 ) ) ;
#32239=CARTESIAN_POINT ( 'NONE',  ( -78.23797558997959811, -294.2994180815049958, -331.4859898249936236 ) ) ;
#32240=CARTESIAN_POINT ( 'NONE',  ( -58.16716152484593749, -275.7833505258702189, -198.2569754551813901 ) ) ;
#32241=CARTESIAN_POINT ( 'NONE',  ( -54.24314367885441612, -274.4806985650496358, -199.2398562268362241 ) ) ;
#32243=CARTESIAN_POINT ( 'NONE',  ( -6.326998723337653452, -286.6668614897027965, -339.0378615201952925 ) ) ;
#32244=CARTESIAN_POINT ( 'NONE',  ( -65.81118855939183732, -273.5023600684870075, -203.1414167560695319 ) ) ;
#32246=CARTESIAN_POINT ( 'NONE',  ( 36.38539468981196023, -287.8314402785017023, -292.6176190156853067 ) ) ;
#32247=CARTESIAN_POINT ( 'NONE',  ( -34.15967351294457899, -300.0716840673962338, -195.0048420694594711 ) ) ;
#32248=CARTESIAN_POINT ( 'NONE',  ( -106.4456722396703725, -294.9276701827540137, -241.6440592496219608 ) ) ;
#32249=CARTESIAN_POINT ( 'NONE',  ( -38.73988127609003840, -282.2664427798089832, -347.1869203580518501 ) ) ;
#32251=CARTESIAN_POINT ( 'NONE',  ( -111.3836069725953024, -276.3945524031435070, -282.6228425162307758 ) ) ;
#32254=CARTESIAN_POINT ( 'NONE',  ( -101.4631401186011459, -289.8340395935156266, -234.5416235684411106 ) ) ;
#32257=CARTESIAN_POINT ( 'NONE',  ( -73.57132889767861172, -289.5716214838470819, -204.6337891756796523 ) ) ;
#32258=CARTESIAN_POINT ( 'NONE',  ( 7.739928421113376089, -276.2007600089746120, -212.0657106346083083 ) ) ;
#32259=CARTESIAN_POINT ( 'NONE',  ( 37.29393907335293079, -283.1845464576910558, -286.7962111365069973 ) ) ;
#32260=CARTESIAN_POINT ( 'NONE',  ( 95.58944840416511113, -297.7283352241495891, -195.0504912288055550 ) ) ;
#32261=CARTESIAN_POINT ( 'NONE',  ( -32.14570100355977189, -282.9847833372272135, -343.1759625755273078 ) ) ;
#32262=CARTESIAN_POINT ( 'NONE',  ( -27.22700639542446055, -275.6083583574713884, -197.4190153406925958 ) ) ;
#32263=CARTESIAN_POINT ( 'NONE',  ( 35.26764813401671717, -276.4783980577627176, -279.7369091912106001 ) ) ;
#32264=CARTESIAN_POINT ( 'NONE',  ( 26.61322196549786412, -284.0789346999468421, -309.6357126892287965 ) ) ;
#32267=CARTESIAN_POINT ( 'NONE',  ( 34.45072584340250188, -293.7381287420843705, -298.1972020753325410 ) ) ;
#32268=CARTESIAN_POINT ( 'NONE',  ( -70.74050075527206616, -287.5893880694603126, -203.5908323389459156 ) ) ;
#32270=CARTESIAN_POINT ( 'NONE',  ( -72.02372285203398405, -283.1237833571631768, -198.2697987213421698 ) ) ;
#32271=CARTESIAN_POINT ( 'NONE',  ( -110.5160414611179505, -277.4519852121095482, -293.9776425699749325 ) ) ;
#32272=CARTESIAN_POINT ( 'NONE',  ( -110.0250025524820785, -288.6594980502424619, -293.4154749958042885 ) ) ;
#32273=CARTESIAN_POINT ( 'NONE',  ( -72.72374852345218699, -287.0947370963862681, -205.7029838738236265 ) ) ;
#32274=CARTESIAN_POINT ( 'NONE',  ( 6.008198648516186680, -278.2156342905747124, -330.4140878174021054 ) ) ;
#32275=CARTESIAN_POINT ( 'NONE',  ( -32.36307777113534456, -287.5390106590699588, -194.0996451132782283 ) ) ;
#32276=CARTESIAN_POINT ( 'NONE',  ( 23.44754035571330775, -284.1506537678160953, -314.3111134739431236 ) ) ;
#32277=CARTESIAN_POINT ( 'NONE',  ( -14.58766863316399309, -276.9319815117594317, -343.9781706223171796 ) ) ;
#32278=CARTESIAN_POINT ( 'NONE',  ( -102.0981396277692852, -277.8377682362244059, -312.1189909655019505 ) ) ;
#32280=CARTESIAN_POINT ( 'NONE',  ( -107.1648759016839847, -298.8115035065173970, -244.4045847718304572 ) ) ;
#32282=CARTESIAN_POINT ( 'NONE',  ( -112.3452863284742875, -275.1604526064900824, -261.9424758988611188 ) ) ;
#32283=CARTESIAN_POINT ( 'NONE',  ( -36.88194192547111072, -296.1974401242884483, -194.5964544069025806 ) ) ;
#32286=CARTESIAN_POINT ( 'NONE',  ( -89.13386536462138565, -277.3122977515685648, -321.9650924524983111 ) ) ;
#32287=AXIS2_PLACEMENT_3D ( 'NONE', #32110, #75657, #54341 ) ;
#32288=CARTESIAN_POINT ( 'NONE',  ( -69.97662454651160147, -274.8369238568205901, -201.0433116877852626 ) ) ;
#32289=CARTESIAN_POINT ( 'NONE',  ( 38.63666777377471817, -280.7483853767105870, -281.3204894922679387 ) ) ;
#32290=CARTESIAN_POINT ( 'NONE',  ( 36.28010480961432904, -289.2133780135225720, -262.7582336555315692 ) ) ;
#32291=CARTESIAN_POINT ( 'NONE',  ( -112.2122030526331287, -298.2590715771484042, -255.5589953414583704 ) ) ;
#32292=CARTESIAN_POINT ( 'NONE',  ( -44.74191011189814304, -296.3487757258884017, -346.6588917906612437 ) ) ;
#32293=CARTESIAN_POINT ( 'NONE',  ( 9.989181565077073444, -294.7057653998595015, -212.3300037107543972 ) ) ;
#32294=CARTESIAN_POINT ( 'NONE',  ( -38.35368219736916728, -278.0392828269668257, -195.5219115804316061 ) ) ;
#32296=CARTESIAN_POINT ( 'NONE',  ( 33.33626291598083213, -283.1662259193070099, -246.8334676036583915 ) ) ;
#32297=CARTESIAN_POINT ( 'NONE',  ( -37.80746338938782714, -296.1261205785993980, -195.9225710704702124 ) ) ;
#32298=CARTESIAN_POINT ( 'NONE',  ( -110.3357146914367490, -285.8744170749661748, -292.2767830340557680 ) ) ;
#32299=CARTESIAN_POINT ( 'NONE',  ( -4.443570321141995016, -285.4166419349108992, -204.8482251309627031 ) ) ;
#32300=CARTESIAN_POINT ( 'NONE',  ( -82.07967447956953322, -220.3963648522054370, -351.9527955420491594 ) ) ;
#32303=CARTESIAN_POINT ( 'NONE',  ( 33.41010517135428159, -286.9799189786174338, -252.2477048155458021 ) ) ;
#32305=CARTESIAN_POINT ( 'NONE',  ( -92.20297315227257684, -284.8937206349091866, -323.9496730260005961 ) ) ;
#32307=CARTESIAN_POINT ( 'NONE',  ( 0.6198357200240276477, -274.9067993234393157, -207.9831628796951861 ) ) ;
#32308=CARTESIAN_POINT ( 'NONE',  ( 34.48725945327707620, -286.0087922681374835, -243.7414019185382585 ) ) ;
#32309=CONICAL_SURFACE ( 'NONE', #41410, 6.249455242036738412, 0.09862129276975223346 ) ;
#32310=CARTESIAN_POINT ( 'NONE',  ( -44.85303184136727594, -290.8796471091947637, -193.9862463122042016 ) ) ;
#32313=CARTESIAN_POINT ( 'NONE',  ( -97.16550227132226780, -280.7118629999972654, -222.9921360119068368 ) ) ;
#32314=CARTESIAN_POINT ( 'NONE',  ( 34.56926708955342775, -282.2332892996662963, -297.8303204697812134 ) ) ;
#32315=CARTESIAN_POINT ( 'NONE',  ( -21.33282851196157992, -277.7666405000204577, -200.3683826091710216 ) ) ;
#32316=CARTESIAN_POINT ( 'NONE',  ( -99.42433144932330435, -248.5360940272530001, -334.3804182888130754 ) ) ;
#32318=CARTESIAN_POINT ( 'NONE',  ( 36.16979982627429280, -277.3721129016309419, -256.3579824915490804 ) ) ;
#32319=CARTESIAN_POINT ( 'NONE',  ( 173.1255004754493712, 243.5021256030123027, -179.3842541629520611 ) ) ;
#32321=CARTESIAN_POINT ( 'NONE',  ( 14.49507151843468300, -278.8053531906564331, -216.5787671083034240 ) ) ;
#32322=CARTESIAN_POINT ( 'NONE',  ( -70.34718550594215003, -297.2412399472815423, -338.8196606254690550 ) ) ;
#32323=CARTESIAN_POINT ( 'NONE',  ( -88.19069716722290764, -296.6661121821695133, -217.7711979766835384 ) ) ;
#32324=CARTESIAN_POINT ( 'NONE',  ( -25.02510931891547230, -291.7128637054604496, -194.4148969184278712 ) ) ;
#32326=CARTESIAN_POINT ( 'NONE',  ( -113.6465790904518229, -295.0648493868808373, -275.2831899912055178 ) ) ;
#32327=CARTESIAN_POINT ( 'NONE',  ( 15.61761637174408079, -285.2169997241592796, -218.9631490465316119 ) ) ;
#32328=CARTESIAN_POINT ( 'NONE',  ( 23.96626899298357571, -295.9863589187013986, -312.3103182508652935 ) ) ;
#32329=CARTESIAN_POINT ( 'NONE',  ( 18.13753566622487057, -288.1847579160051396, -222.1605176268522257 ) ) ;
#32331=CARTESIAN_POINT ( 'NONE',  ( 34.23643443135534170, -294.8458823230296844, -298.0990138190774132 ) ) ;
#32332=CARTESIAN_POINT ( 'NONE',  ( -109.9331421419225308, -284.9296889926879999, -279.0719114223929864 ) ) ;
#32333=CARTESIAN_POINT ( 'NONE',  ( -39.11411323897724657, -293.8688619392580108, -346.9435394099575660 ) ) ;
#32335=CARTESIAN_POINT ( 'NONE',  ( -92.70285612861634661, -292.0866334253823311, -217.0003165465266477 ) ) ;
#32336=CARTESIAN_POINT ( 'NONE',  ( -79.56588751481959321, -291.9908621514224478, -205.9806751378311560 ) ) ;
#32337=CARTESIAN_POINT ( 'NONE',  ( -29.17101451503082998, -289.1124041353048710, -342.9024158832058333 ) ) ;
#32339=LINE ( 'NONE', #61240, #86626 ) ;
#32340=CARTESIAN_POINT ( 'NONE',  ( -111.6566287797313066, -274.6499668381442234, -256.4209244867586790 ) ) ;
#32341=CARTESIAN_POINT ( 'NONE',  ( -108.7906646557815122, -271.7004588130334923, -242.5917494710402309 ) ) ;
#32343=CARTESIAN_POINT ( 'NONE',  ( 35.66252737393860173, -280.6953467798653037, -276.7836653902211879 ) ) ;
#32346=CARTESIAN_POINT ( 'NONE',  ( 38.43259605435577697, -274.8919769162088187, -256.9522760687449363 ) ) ;
#32347=CARTESIAN_POINT ( 'NONE',  ( -108.5001396552410284, -295.2833197611125797, -251.1504883938874855 ) ) ;
#32348=CARTESIAN_POINT ( 'NONE',  ( -73.42196341943370896, -279.3965083370046614, -335.2531643537352011 ) ) ;
#32349=CARTESIAN_POINT ( 'NONE',  ( 31.32626742168720568, -273.3184131282981753, -242.0200803012417055 ) ) ;
#32350=CARTESIAN_POINT ( 'NONE',  ( -109.1708914671404216, -297.9559892846735352, -255.2109676722522522 ) ) ;
#32351=CARTESIAN_POINT ( 'NONE',  ( -75.38275588740876287, -298.6120167188104233, -207.6356462301342276 ) ) ;
#32352=CARTESIAN_POINT ( 'NONE',  ( -59.93058115945312636, -299.3644882323160914, -197.5312893871767983 ) ) ;
#32353=CARTESIAN_POINT ( 'NONE',  ( -27.19254136597337279, -272.2005099159476345, -195.6402176614799941 ) ) ;
#32354=CARTESIAN_POINT ( 'NONE',  ( 35.74420764866165001, -294.2447221213153625, -273.4850649989338649 ) ) ;
#32355=CARTESIAN_POINT ( 'NONE',  ( -3.348062670835536991, -291.0850095665383037, -205.0939169477127848 ) ) ;
#32357=CARTESIAN_POINT ( 'NONE',  ( 39.25541075472718688, -275.9471107175803581, -262.5803281006356542 ) ) ;
#32358=CARTESIAN_POINT ( 'NONE',  ( -102.0314305036114177, -273.1804833387137705, -236.4250285445152713 ) ) ;
#32359=CARTESIAN_POINT ( 'NONE',  ( 36.26447050974762476, -283.7390765580696552, -286.5620009352759894 ) ) ;
#32360=CARTESIAN_POINT ( 'NONE',  ( -65.08904940218464219, -282.0920310978439147, -341.6730784576504902 ) ) ;
#32362=CARTESIAN_POINT ( 'NONE',  ( -82.90325194787516239, -282.8907312274963601, -327.6690081599109021 ) ) ;
#32363=CARTESIAN_POINT ( 'NONE',  ( -93.05776711153009728, -281.8497423675445361, -320.8356247917740802 ) ) ;
#32364=CARTESIAN_POINT ( 'NONE',  ( 29.68352570831852333, -274.5330799555257499, -300.7419345787084808 ) ) ;
#32365=CARTESIAN_POINT ( 'NONE',  ( -32.04088924950214334, -282.1190584623532800, -195.4975217166891355 ) ) ;
#32368=CARTESIAN_POINT ( 'NONE',  ( -5.430534733744966758, -272.8648975631196549, -201.1648901865350183 ) ) ;
#32370=CARTESIAN_POINT ( 'NONE',  ( -106.9488764411532600, -280.1831986199911171, -298.7313388095516302 ) ) ;
#32372=CARTESIAN_POINT ( 'NONE',  ( -109.5571685140269551, -286.7588443331821395, -247.9533079844526640 ) ) ;
#32375=CARTESIAN_POINT ( 'NONE',  ( -69.34226144694790150, -289.6310272311670815, -202.5168244816508150 ) ) ;
#32377=CARTESIAN_POINT ( 'NONE',  ( -108.2150961877190838, -295.5983150738486529, -251.2315247105417200 ) ) ;
#32378=CARTESIAN_POINT ( 'NONE',  ( -91.51002333266008293, -287.9728055004209750, -321.1970073512915747 ) ) ;
#32380=CARTESIAN_POINT ( 'NONE',  ( -111.1138956086464020, -294.3775424377677723, -283.9477102097837928 ) ) ;
#32381=CARTESIAN_POINT ( 'NONE',  ( 11.64741596629121823, -285.1973680554068551, -211.7876736251588738 ) ) ;
#32382=CARTESIAN_POINT ( 'NONE',  ( 27.56825487165307820, -283.6262049400421006, -305.4771848922749200 ) ) ;
#32383=CARTESIAN_POINT ( 'NONE',  ( 6.324130911590088111, -280.7083881226946005, -332.6128191718094058 ) ) ;
#32384=CARTESIAN_POINT ( 'NONE',  ( -13.28787469182305792, -288.7308308813364874, -339.2843613905860707 ) ) ;
#32385=AXIS2_PLACEMENT_3D ( 'NONE', #74700, #67137, #2271 ) ;
#32386=CARTESIAN_POINT ( 'NONE',  ( 32.53038872741445431, -282.6714239488571820, -247.1080796639563744 ) ) ;
#32387=CARTESIAN_POINT ( 'NONE',  ( -34.31686453079056776, -280.8939502873100196, -197.2496267091526363 ) ) ;
#32388=CARTESIAN_POINT ( 'NONE',  ( 33.30329505202329443, -289.1932470475849186, -244.1372460893867071 ) ) ;
#32389=CARTESIAN_POINT ( 'NONE',  ( -85.21807702622959368, -297.5780897807170504, -210.0547954318478503 ) ) ;
#32392=CARTESIAN_POINT ( 'NONE',  ( -32.68260308280422066, -274.1093157272443932, -193.4890523665611113 ) ) ;
#32393=CARTESIAN_POINT ( 'NONE',  ( -9.128663604227064354, -294.4026341400522142, -201.1984510684911527 ) ) ;
#32395=CARTESIAN_POINT ( 'NONE',  ( -4.771743288812468897, -279.1233781216988064, -337.9199732462171255 ) ) ;
#32397=CARTESIAN_POINT ( 'NONE',  ( -34.38922664861754441, -275.0149512517467656, -345.4697814598350192 ) ) ;
#32399=CARTESIAN_POINT ( 'NONE',  ( -96.71010705810103047, -295.5989722807323687, -222.5925856902501039 ) ) ;
#32400=CARTESIAN_POINT ( 'NONE',  ( -76.61200643603298488, -272.8598460136507242, -208.7029010885975993 ) ) ;
#32401=CARTESIAN_POINT ( 'NONE',  ( -95.67497020326675283, -292.7002995774033138, -225.3284925121474771 ) ) ;
#32403=CARTESIAN_POINT ( 'NONE',  ( -34.78945241426409751, -284.7798300885380627, -344.3430452014534922 ) ) ;
#32404=CARTESIAN_POINT ( 'NONE',  ( -97.89255279504368445, -292.6043255270955115, -223.7330670399650501 ) ) ;
#32405=CARTESIAN_POINT ( 'NONE',  ( 1.435608388423053272, -293.8737294512537801, -204.3489427776735852 ) ) ;
#32406=CARTESIAN_POINT ( 'NONE',  ( 35.70797416219151899, -293.3907598458124539, -270.7620413100024734 ) ) ;
#32407=CARTESIAN_POINT ( 'NONE',  ( 21.90533250431893819, -288.9218133125194186, -224.3742744604433597 ) ) ;
#32408=CARTESIAN_POINT ( 'NONE',  ( 21.96934963379798589, -281.0587317681415129, -221.2571529626713414 ) ) ;
#32409=CARTESIAN_POINT ( 'NONE',  ( -95.42056359907546437, -293.9693401420921646, -318.7150820059781609 ) ) ;
#32410=CARTESIAN_POINT ( 'NONE',  ( -47.25846401018586818, -283.0081704693097890, -346.7198620699309117 ) ) ;
#32411=CARTESIAN_POINT ( 'NONE',  ( 31.81112822514513994, -277.9017789624232364, -298.6009576284413924 ) ) ;
#32412=CARTESIAN_POINT ( 'NONE',  ( -53.88499642491207453, -275.4017514920610097, -344.3515122700736129 ) ) ;
#32414=CARTESIAN_POINT ( 'NONE',  ( -93.47337082312604650, -283.3967610902026877, -317.1288845192268013 ) ) ;
#32415=CARTESIAN_POINT ( 'NONE',  ( -74.82709311628362059, -280.7695548127976508, -203.5565220971852796 ) ) ;
#32416=CARTESIAN_POINT ( 'NONE',  ( 24.52078660090812434, -286.0053344338332977, -224.9094629061029593 ) ) ;
#32417=CARTESIAN_POINT ( 'NONE',  ( -9.364938622540815771, -294.1829186509569354, -201.7845193528349910 ) ) ;
#32418=CARTESIAN_POINT ( 'NONE',  ( 27.80787594902894355, -276.6297915557126430, -230.7384826736917773 ) ) ;
#32419=CARTESIAN_POINT ( 'NONE',  ( 36.02534764677034218, -277.1417454587772227, -292.1001054445010823 ) ) ;
#32420=CARTESIAN_POINT ( 'NONE',  ( -108.7652147455494003, -278.1864210546953586, -285.4502387065083440 ) ) ;
#32421=CARTESIAN_POINT ( 'NONE',  ( -44.77594189955190274, -299.9581344516384434, -195.8463219659928427 ) ) ;
#32422=CARTESIAN_POINT ( 'NONE',  ( -65.76657831342915017, -283.6794743276750523, -201.0813000019735739 ) ) ;
#32423=CARTESIAN_POINT ( 'NONE',  ( -44.89074754434063408, -291.6259169909620255, -193.7004026931768692 ) ) ;
#32424=CARTESIAN_POINT ( 'NONE',  ( -74.02413100341306063, -291.1311924263224000, -337.1655309676206116 ) ) ;
#32425=CARTESIAN_POINT ( 'NONE',  ( -41.59709081642525774, -290.9177642364082885, -197.1255578693039752 ) ) ;
#32427=CARTESIAN_POINT ( 'NONE',  ( -4.838180963169321558, -291.0466057699269413, -201.2081893590344635 ) ) ;
#32428=CARTESIAN_POINT ( 'NONE',  ( -7.257658260007986861, -292.1246974259365174, -203.8251283849321851 ) ) ;
#32430=CARTESIAN_POINT ( 'NONE',  ( -41.72907601921568244, -290.1858438987486011, -346.9395758839061727 ) ) ;
#32431=CARTESIAN_POINT ( 'NONE',  ( -85.55762702215886861, -280.0154206062724143, -215.4146252681086366 ) ) ;
#32432=CARTESIAN_POINT ( 'NONE',  ( -113.2937005686993501, -295.6070294040862905, -259.6461614683297512 ) ) ;
#32433=CARTESIAN_POINT ( 'NONE',  ( 1.463067592329282629, -287.2078707335562626, -203.9567746776621391 ) ) ;
#32435=CARTESIAN_POINT ( 'NONE',  ( 1.507341928917059759, -286.8897900295468162, -203.8890598430689636 ) ) ;
#32436=CARTESIAN_POINT ( 'NONE',  ( -76.13476189213297118, -283.9191052613003308, -332.2851683735178767 ) ) ;
#32437=CARTESIAN_POINT ( 'NONE',  ( 173.7950248217412081, 243.4804843829244589, -179.6775006142443374 ) ) ;
#32438=CARTESIAN_POINT ( 'NONE',  ( 23.88957826587596855, -22.54207381367533714, -343.5632202908770978 ) ) ;
#32439=CARTESIAN_POINT ( 'NONE',  ( -55.84047289447126872, -169.3153992383580260, -360.5835854410441925 ) ) ;
#32440=CARTESIAN_POINT ( 'NONE',  ( -71.73912590187161697, -276.7161221966420044, -334.9462867330391873 ) ) ;
#32441=CARTESIAN_POINT ( 'NONE',  ( 35.32873332832064506, -274.3456371679985182, -260.7053334545656185 ) ) ;
#32442=CARTESIAN_POINT ( 'NONE',  ( -82.92906580391864679, -296.9550300905445397, -208.3165517894283028 ) ) ;
#32443=CARTESIAN_POINT ( 'NONE',  ( 202.5199829828008546, 289.9242760918802446, -82.50643157239619541 ) ) ;
#32444=CARTESIAN_POINT ( 'NONE',  ( -97.55124454307568271, -276.6019314941992207, -317.5639678570206570 ) ) ;
#32445=CARTESIAN_POINT ( 'NONE',  ( -97.11280006326180114, -274.9161399701190476, -226.6251671795039897 ) ) ;
#32446=CARTESIAN_POINT ( 'NONE',  ( -110.3674973873447982, -290.9976182341925437, -273.9181996503078267 ) ) ;
#32447=CARTESIAN_POINT ( 'NONE',  ( -99.79627983481546494, -297.9493676950479539, -225.5997027414165927 ) ) ;
#32448=CARTESIAN_POINT ( 'NONE',  ( -105.2022907227369899, -297.5146665670653192, -233.9925021789906623 ) ) ;
#32449=CARTESIAN_POINT ( 'NONE',  ( -70.92890994336237043, -295.6748925296958532, -335.1894473489932693 ) ) ;
#32452=CARTESIAN_POINT ( 'NONE',  ( -72.15505482187559494, -279.4290425871595289, -337.4377885480166697 ) ) ;
#32455=CARTESIAN_POINT ( 'NONE',  ( 22.47146288680990267, -281.7094525246209855, -318.7752120679950281 ) ) ;
#32456=CARTESIAN_POINT ( 'NONE',  ( -94.62961870973823864, -278.8509340769741129, -316.0046354399279949 ) ) ;
#32457=CARTESIAN_POINT ( 'NONE',  ( 37.19283742599328235, -277.4996523657072203, -285.1454586091329020 ) ) ;
#32458=CARTESIAN_POINT ( 'NONE',  ( -105.0087371295930438, -271.4220887925192756, -241.0448966601455822 ) ) ;
#32460=CARTESIAN_POINT ( 'NONE',  ( -109.9037758266207447, -278.6076168075037458, -278.7919245255241094 ) ) ;
#32461=CARTESIAN_POINT ( 'NONE',  ( -92.06125906436095363, -274.0974753519782325, -216.4173631066185521 ) ) ;
#32463=CARTESIAN_POINT ( 'NONE',  ( 38.85478441651682147, -286.3236334001359751, -277.2454490988039879 ) ) ;
#32464=CARTESIAN_POINT ( 'NONE',  ( -64.20806928646177880, -275.7018206846278190, -200.3244534211798111 ) ) ;
#32465=CARTESIAN_POINT ( 'NONE',  ( 38.34306530093780907, -273.9944500992896224, -259.8529033564357746 ) ) ;
#32467=CARTESIAN_POINT ( 'NONE',  ( -101.7902247573781835, -289.2768991933272673, -305.0949833633569028 ) ) ;
#32469=CARTESIAN_POINT ( 'NONE',  ( -101.3389253635708940, -283.3377889204409712, -313.0907938094499627 ) ) ;
#32470=CARTESIAN_POINT ( 'NONE',  ( 35.33347399751815487, -279.6088476364748203, -256.2837836662665154 ) ) ;
#32472=CARTESIAN_POINT ( 'NONE',  ( 29.84507023166866091, -280.5294049156908613, -300.5080369959069913 ) ) ;
#32473=CARTESIAN_POINT ( 'NONE',  ( -99.29217534005471180, -283.1938932173042645, -229.0882113862969334 ) ) ;
#32474=CARTESIAN_POINT ( 'NONE',  ( -77.32257694246789015, -291.5880538007035625, -333.8761119678735554 ) ) ;
#32475=CARTESIAN_POINT ( 'NONE',  ( -79.29432953402132966, -280.6766997171642970, -210.1356467112776727 ) ) ;
#32476=CARTESIAN_POINT ( 'NONE',  ( -108.0627254117779188, -262.2579384450284010, -317.5737540118648781 ) ) ;
#32477=CARTESIAN_POINT ( 'NONE',  ( 36.56041673708003970, -279.7172213550786068, -251.7891622266978402 ) ) ;
#32478=CARTESIAN_POINT ( 'NONE',  ( -6.727252182799131397, -294.4541666521365642, -201.8800124452416185 ) ) ;
#32479=CARTESIAN_POINT ( 'NONE',  ( -72.02403946465955187, -277.8398574152951142, -202.7366815037724450 ) ) ;
#32480=CARTESIAN_POINT ( 'NONE',  ( -37.80208646944788597, -277.7094474323222926, -343.4740720598367147 ) ) ;
#32481=CARTESIAN_POINT ( 'NONE',  ( -27.58423511042995102, -284.9287777058946176, -344.9438766267732603 ) ) ;
#32483=CARTESIAN_POINT ( 'NONE',  ( -74.92579139469680172, -291.4687874365460516, -335.9107196758862415 ) ) ;
#32484=CARTESIAN_POINT ( 'NONE',  ( 14.14627780109534427, -285.9504403143811260, -213.2533595926338990 ) ) ;
#32485=CARTESIAN_POINT ( 'NONE',  ( -91.33068523627710533, -289.6678765267430435, -220.0271344497617179 ) ) ;
#32487=CARTESIAN_POINT ( 'NONE',  ( 34.31833529681122030, -274.0225722704693112, -253.9927497677400083 ) ) ;
#32488=CARTESIAN_POINT ( 'NONE',  ( 15.17361440809236051, -292.4412160138317063, -322.9024775557434168 ) ) ;
#32491=CARTESIAN_POINT ( 'NONE',  ( 32.69576719977037982, -291.6425581746654530, -240.0715005980366357 ) ) ;
#32492=CARTESIAN_POINT ( 'NONE',  ( -111.1095757517718425, -286.1806999290394060, -268.1837482222301219 ) ) ;
#32493=CARTESIAN_POINT ( 'NONE',  ( 11.74394287517603352, -286.6211308050484377, -328.3660631366237226 ) ) ;
#32494=CARTESIAN_POINT ( 'NONE',  ( 2.752976485267746298, -288.0270291713399047, -208.6538102823708698 ) ) ;
#32496=CARTESIAN_POINT ( 'NONE',  ( 23.66306833262262188, -287.7947908036791773, -229.8835274948197025 ) ) ;
#32497=CARTESIAN_POINT ( 'NONE',  ( -17.09334165656645510, -294.2922010771532655, -197.7772989917731650 ) ) ;
#32498=CARTESIAN_POINT ( 'NONE',  ( -97.66878104912215974, -276.0143579469335577, -315.8791474220496411 ) ) ;
#32500=CARTESIAN_POINT ( 'NONE',  ( -112.7720585040347743, -278.6924352973895793, -285.7887082993948979 ) ) ;
#32501=CARTESIAN_POINT ( 'NONE',  ( -37.76201442796587315, -290.1267778830119255, -194.8022830366007554 ) ) ;
#32502=CARTESIAN_POINT ( 'NONE',  ( -73.76564290355869957, -279.5822535842049774, -202.5059403146675265 ) ) ;
#32503=CARTESIAN_POINT ( 'NONE',  ( -55.72254121264094096, -299.7944200614800820, -197.9612934927405377 ) ) ;
#32505=CARTESIAN_POINT ( 'NONE',  ( -110.0379128990311699, -282.3150227119010083, -288.8072910518047252 ) ) ;
#32507=CARTESIAN_POINT ( 'NONE',  ( -110.7164920681103411, -276.5455406390557300, -281.6307847316989523 ) ) ;
#32508=CARTESIAN_POINT ( 'NONE',  ( 22.63986663616999451, -280.1672660035160334, -315.3856923870417290 ) ) ;
#32509=DIRECTION ( 'NONE',  ( 0.000000000000000000, 0.000000000000000000, -1.000000000000000000 ) ) ;
#32510=CARTESIAN_POINT ( 'NONE',  ( 29.92266606438576559, -274.5032344958930253, -306.5033545522953773 ) ) ;
#32512=CARTESIAN_POINT ( 'NONE',  ( -95.30691719897633618, -297.4365997791711607, -315.8665172726256287 ) ) ;
#32513=CARTESIAN_POINT ( 'NONE',  ( 23.99955774836108091, -281.0876062262976234, -316.3909191206939227 ) ) ;
#32514=CARTESIAN_POINT ( 'NONE',  ( -75.34295520402633883, -298.4736196271046538, -207.6979000982530579 ) ) ;
#32515=CARTESIAN_POINT ( 'NONE',  ( -35.50359419720567189, -299.3898790440853759, -193.8538639921639799 ) ) ;
#32516=CARTESIAN_POINT ( 'NONE',  ( -35.38550754078937643, -273.7440612112474128, -197.3536722973015856 ) ) ;
#32517=CARTESIAN_POINT ( 'NONE',  ( 36.88353150890747401, -295.4142531733328951, -259.6086467588099822 ) ) ;
#32518=CARTESIAN_POINT ( 'NONE',  ( 26.35617176857961041, -287.1481718986930787, -227.0757909323515378 ) ) ;
#32519=( BOUNDED_SURFACE ( )  B_SPLINE_SURFACE ( 3, 2, ( 
 ( #22482, #22944, #93514, #64688, #14478, #51817, #86881, #35775, #58947, #87795, #64228, #71778, #72233, #15860, #65613, #28672, #65147, #44719, #28214, #57102, #51356, #50904, #248, #80246, #21093, #36229, #57557, #49963, #86402, #21556, #29131, #7347, #7804, #50440, #58027, #44247, #79788, #725, #22035, #15383, #66069, #14930, #43785, #29611, #73157, #58489, #8280, #37160, #1181, #30062, #80710, #47030, #81629, #16316, #17256, #45630, #74537, #1639, #68373, #46115, #31462, #9669, #16776, #37607, #67455, #53704, #38552, #60351, #3503, #23879, #38997, #75018, #2583, #23427, #89188, #10131, #66520, #82571, #67909, #24341, #74070, #30519, #45168, #53216, #52747, #82096, #81172, #3035, #66976, #31918, #89651, #46574, #60810, #59417, #24821, #9189, #17719, #38067, #75472, #2115, #10595, #39456, #32395, #61294, #88731, #88271, #90129, #31005, #59891, #25280, #54157, #83026, #18180, #8731, #52293, #84894, #12005, #56041, #70722, #20533, #33788, #91533, #75933 ),
 ( #70264, #56527, #41811, #40855, #48924, #92000, #90573, #62703, #5854, #34263, #61741, #68848, #55104, #12973, #26690, #32852, #39931, #55579, #69773, #34725, #84427, #63170, #3977, #19575, #27153, #63641, #18644, #4903, #40386, #20044, #77345, #11061, #83486, #25733, #48443, #92463, #54615, #83971, #47511, #12479, #19119, #47974, #76417, #27628, #41329, #5398, #76878, #77823, #11539, #85384, #69304, #4432, #33312, #62208, #91038, #26210, #21925, #43229, #64111, #28562, #50798, #78293, #29500, #86763, #72129, #20985, #42278, #56996, #50321, #64585, #141, #28109, #93410, #13892, #79682, #36582, #87225, #57453, #71191, #29021, #49852, #79227, #78751, #65496, #42746, #22372, #80135, #36121, #51246, #35670, #6318, #86295, #71662, #6795, #21448, #14369, #1073, #7245, #8167, #65038, #58381, #57908, #15275, #44133, #87682, #14825, #43679, #49403, #72575, #7697, #615, #73038, #37051, #92949, #13431, #65962, #35186, #85834, #29953, #58837, #73510, #61176, #60236 ),
 ( #80590, #37950, #8620, #45999, #81977, #15746, #67340, #89537, #81512, #22834, #51702, #23767, #81061, #37497, #44606, #73956, #52632, #88620, #89074, #9071, #16659, #31805, #2471, #24223, #66406, #1522, #53099, #30409, #52179, #66858, #17133, #45514, #16206, #82459, #17607, #74904, #74415, #39341, #23305, #10016, #38886, #1993, #9545, #45057, #67795, #31348, #59300, #30885, #59778, #68260, #38431, #2920, #88148, #3382, #60698, #24701, #53585, #46458, #75360, #10475, #32270, #27038, #90924, #5740, #40740, #3863, #91419, #54041, #90464, #26090, #5281, #34614, #62091, #33667, #11890, #84311, #70613, #55927, #54979, #63055, #12359, #10944, #47860, #84779, #48328, #75820, #82911, #69193, #19930, #69657, #46918, #18065, #4787, #83855, #48798, #62577, #77230, #39810, #26572, #77708, #68732, #4323, #12857, #41695, #19007, #76763, #32742, #55460, #41207, #19462, #83374, #91884, #25621, #70145, #61631, #54503, #40277, #34150, #18523, #47389, #90012, #25167, #76299 ),
 ( #11425, #33200, #87121, #22271, #8055, #42158, #13783, #44028, #35, #6207, #93303, #72928, #56406, #63525, #50693, #79114, #28453, #79578, #72473, #85267, #35075, #50210, #42634, #13318, #15170, #85728, #51145, #71550, #7589, #57348, #43575, #58279, #92352, #21340, #14262, #27510, #27996, #64934, #6685, #86653, #21818, #71075, #20416, #14722, #49284, #63992, #35562, #78180, #92833, #56888, #7142, #20874, #64475, #49746, #80029, #78643, #86188, #43120, #36475, #28915, #72026, #36016, #65391, #57803, #504, #29386, #37850, #1418, #51595, #65860, #88038, #66756, #8972, #9437, #23195, #1884, #45893, #81408, #74311, #87576, #24120, #67692, #73406, #30777, #30304, #81873, #38324, #968, #44500, #58731, #67238, #24586, #75255, #16103, #8516, #45412, #73855, #59676, #29848, #2820, #2368, #88519, #23667, #44955, #22720, #52533, #17024, #16558, #31246, #31702, #52076, #60133, #88972, #52999, #80481, #74798, #9915, #15631, #38788, #60595, #89430, #37395, #66304 ),
 ( #53474, #82353, #17501, #46354, #59192, #36947, #80959, #83268, #90815, #39697, #69545, #18897, #32165, #68622, #18412, #26926, #47272, #76650, #46810, #55814, #76188, #61528, #55352, #11318, #61980, #62941, #12246, #84204, #5163, #48685, #25974, #54858, #10370, #3756, #11775, #40169, #33549, #62457, #53937, #39237, #91300, #68153, #82806, #54395, #61066, #89907, #3273, #47752, #25065, #69086, #32638, #34038, #17957, #25516, #75712, #26463, #4675, #10835, #83740, #77117, #4214, #90359, #33089, #40627, #19351, #48213, #41092, #70020, #91775, #84668, #19819, #34966, #13670, #86532, #28343, #21226, #34506, #64821, #14606, #20303, #42520, #42047, #28805, #78989, #12740, #85150, #5631, #50095, #65276, #22161, #56776, #49174, #86075, #20764, #49636, #70504, #43464, #14144, #6567, #78531, #85618, #41582, #71432, #57689, #35446, #64365, #72361, #92716, #43008, #71912, #93191, #92242, #57233, #7033, #63413, #21700, #35903, #93645, #78068, #27397, #13211, #50577, #27886 ),
 ( #79472, #7478, #36363, #381, #56287, #29269, #70961, #58165, #6094, #87009, #63878, #77589, #83043, #37737, #54174, #37285, #43916, #66191, #22608, #8407, #44385, #51952, #3994, #15512, #11081, #59079, #60021, #80843, #8859, #18196, #9320, #36830, #72811, #30190, #47048, #1771, #7936, #15054, #30655, #44844, #75949, #66645, #38203, #65749, #59556, #39948, #858, #87922, #68864, #32869, #73747, #88406, #29739, #16446, #67117, #74203, #73295, #61757, #80371, #15992, #58620, #51483, #1308, #45298, #87461, #23073, #90589, #2251, #51029, #23556, #52425, #81300, #79917, #31135, #90147, #25296, #49417, #64131, #4447, #69788, #6333, #56057, #62224, #55594, #35202, #18662, #25750, #12987, #41347, #84442, #41825, #34739, #47529, #91053, #12494, #4919, #69320, #71206, #47989, #40402, #27168, #11554, #55121, #76893, #84911, #19591, #83987, #85399, #20547, #20058, #48460, #42295, #26228, #48940, #77839, #33806, #70280, #19134, #70736, #34278, #76433, #12021, #62719 ),
 ( #40870, #91549, #26706, #77360, #5413, #54631, #63186, #78307, #92016, #63655, #5870, #92478, #13446, #83503, #27643, #56544, #33327, #57467, #630, #7258, #22387, #51259, #42760, #92965, #80150, #57012, #71680, #43244, #93425, #155, #8183, #8632, #65052, #36595, #14839, #87241, #73523, #58851, #29035, #65974, #15290, #13907, #50813, #87695, #44147, #78766, #85848, #72142, #29966, #43692, #49866, #21001, #72589, #86781, #22847, #7711, #73052, #6811, #65510, #51714, #35685, #36135, #80603, #44621, #21940, #79697, #64600, #58395, #37065, #1085, #86310, #15761, #28577, #57923, #21462, #50336, #29515, #37509, #79243, #14385, #28123, #53599, #54052, #30900, #2006, #16671, #82922, #24235, #37963, #90025, #25178, #10955, #45069, #45527, #46929, #2932, #9084, #2483, #75832, #59312, #66419, #82471, #81992, #31360, #17618, #75373, #88161, #66870, #53112, #74428, #16218, #18076, #88632, #81074, #67807, #52192, #59791, #23780, #31816, #60249, #52644, #32282, #61189 ) ),
 .UNSPECIFIED., .T., .F., .F. ) 
 B_SPLINE_SURFACE_WITH_KNOTS ( ( 4, 3, 4 ),
 ( 3, 2, 2, 2, 2, 2, 2, 2, 2, 2, 2, 2, 2, 2, 2, 2, 2, 2, 2, 2, 2, 2, 2, 2, 2, 2, 2, 2, 2, 2, 2, 2, 2, 2, 2, 2, 2, 2, 2, 2, 2, 2, 2, 2, 2, 2, 2, 2, 2, 2, 2, 2, 2, 2, 2, 2, 2, 2, 2, 2, 2, 3 ),
 ( 0.000000000000000000, 0.5000000000000000000, 1.000000000000000000 ),
 ( -0.05855608392607185297, 0.000000000000000000, 0.01428571428571428527, 0.02857142857142857054, 0.04285714285714285754, 0.05714285714285714107, 0.07142857142857142461, 0.08571428571428571508, 0.1000000000000000056, 0.1142857142857142821, 0.1285714285714285587, 0.1428571428571428492, 0.1571428571428571397, 0.1714285714285714302, 0.1857142857142857206, 0.2000000000000000111, 0.2142857142857142738, 0.2285714285714285643, 0.2428571428571428548, 0.2571428571428571175, 0.2714285714285714080, 0.2857142857142856984, 0.2999999999999999889, 0.3142857142857142794, 0.3285714285714285698, 0.3428571428571428603, 0.3571428571428571508, 0.3714285714285714413, 0.3857142857142857317, 0.4000000000000000222, 0.4142857142857143127, 0.4285714285714285476, 0.4428571428571428381, 0.4571428571428571286, 0.4714285714285714191, 0.4857142857142857095, 0.5000000000000000000, 0.5142857142857142350, 0.5285714285714285809, 0.5428571428571428159, 0.5571428571428571619, 0.5714285714285713969, 0.5857142857142857428, 0.5999999999999999778, 0.6142857142857143238, 0.6285714285714285587, 0.6428571428571429047, 0.6571428571428571397, 0.6714285714285713746, 0.6857142857142857206, 0.6999999999999999556, 0.7142857142857143016, 0.7285714285714285365, 0.7428571428571428825, 0.7571428571428571175, 0.7714285714285714635, 0.7857142857142856984, 0.8000000000000000444, 0.8142857142857142794, 0.8285714285714286254, 0.8428571428571428603, 0.8500000000000000888 ),
 .UNSPECIFIED. ) 
 GEOMETRIC_REPRESENTATION_ITEM ( )  RATIONAL_B_SPLINE_SURFACE ( (
 ( 1.000000000000000000, 1.000000000000000000, 1.000000000000000000, 0.9749279121818236193, 1.000000000000000000, 0.9749279121818236193, 1.000000000000000000, 0.9749279121818236193, 1.000000000000000000, 0.9749279121818236193, 1.000000000000000000, 0.9749279121818236193, 1.000000000000000000, 0.9749279121818236193, 1.000000000000000000, 0.9749279121818236193, 1.000000000000000000, 0.9749279121818236193, 1.000000000000000000, 0.9749279121818236193, 1.000000000000000000, 0.9749279121818236193, 1.000000000000000000, 0.9749279121818236193, 1.000000000000000000, 0.9749279121818236193, 1.000000000000000000, 0.9749279121818236193, 1.000000000000000000, 0.9749279121818236193, 1.000000000000000000, 0.9749279121818236193, 1.000000000000000000, 0.9749279121818236193, 1.000000000000000000, 0.9749279121818236193, 1.000000000000000000, 0.9749279121818236193, 1.000000000000000000, 0.9749279121818236193, 1.000000000000000000, 0.9749279121818236193, 1.000000000000000000, 0.9749279121818236193, 1.000000000000000000, 0.9749279121818236193, 1.000000000000000000, 0.9749279121818236193, 1.000000000000000000, 0.9749279121818236193, 1.000000000000000000, 0.9749279121818236193, 1.000000000000000000, 0.9749279121818236193, 1.000000000000000000, 0.9749279121818236193, 1.000000000000000000, 0.9749279121818236193, 1.000000000000000000, 0.9749279121818236193, 1.000000000000000000, 0.9749279121818236193, 1.000000000000000000, 0.9749279121818236193, 1.000000000000000000, 0.9749279121818236193, 1.000000000000000000, 0.9749279121818236193, 1.000000000000000000, 0.9749279121818236193, 1.000000000000000000, 0.9749279121818236193, 1.000000000000000000, 0.9749279121818236193, 1.000000000000000000, 0.9749279121818236193, 1.000000000000000000, 0.9749279121818236193, 1.000000000000000000, 0.9749279121818236193, 1.000000000000000000, 0.9749279121818236193, 1.000000000000000000, 0.9749279121818236193, 1.000000000000000000, 0.9749279121818236193, 1.000000000000000000, 0.9749279121818236193, 1.000000000000000000, 0.9749279121818236193, 1.000000000000000000, 0.9749279121818236193, 1.000000000000000000, 0.9749279121818236193, 1.000000000000000000, 0.9749279121818236193, 1.000000000000000000, 0.9749279121818236193, 1.000000000000000000, 0.9749279121818236193, 1.000000000000000000, 0.9749279121818236193, 1.000000000000000000, 0.9749279121818236193, 1.000000000000000000, 0.9749279121818236193, 1.000000000000000000, 0.9749279121818236193, 1.000000000000000000, 0.9749279121818236193, 1.000000000000000000, 0.9749279121818236193, 1.000000000000000000, 0.9749279121818236193, 1.000000000000000000, 0.9749279121818236193, 1.000000000000000000, 0.9749279121818236193, 1.000000000000000000, 0.9749279121818236193, 1.000000000000000000, 0.9874639560909115321, 0.9874639560909117542),
 ( 0.3333333333333333703, 0.3333333333333333703, 0.3333333333333333703, 0.3249759707272745768, 0.3333333333333333703, 0.3249759707272745768, 0.3333333333333333703, 0.3249759707272745768, 0.3333333333333333703, 0.3249759707272745768, 0.3333333333333333703, 0.3249759707272745768, 0.3333333333333333703, 0.3249759707272745768, 0.3333333333333333703, 0.3249759707272745768, 0.3333333333333333703, 0.3249759707272745768, 0.3333333333333333703, 0.3249759707272745768, 0.3333333333333333703, 0.3249759707272745768, 0.3333333333333333703, 0.3249759707272745768, 0.3333333333333333703, 0.3249759707272745768, 0.3333333333333333703, 0.3249759707272745768, 0.3333333333333333703, 0.3249759707272745768, 0.3333333333333333703, 0.3249759707272745768, 0.3333333333333333703, 0.3249759707272745768, 0.3333333333333333703, 0.3249759707272745768, 0.3333333333333333703, 0.3249759707272745768, 0.3333333333333333703, 0.3249759707272745768, 0.3333333333333333703, 0.3249759707272745768, 0.3333333333333333703, 0.3249759707272745768, 0.3333333333333333703, 0.3249759707272745768, 0.3333333333333333703, 0.3249759707272745768, 0.3333333333333333703, 0.3249759707272745768, 0.3333333333333333703, 0.3249759707272745768, 0.3333333333333333703, 0.3249759707272745768, 0.3333333333333333703, 0.3249759707272745768, 0.3333333333333333703, 0.3249759707272745768, 0.3333333333333333703, 0.3249759707272745768, 0.3333333333333333703, 0.3249759707272745768, 0.3333333333333333703, 0.3249759707272745768, 0.3333333333333333703, 0.3249759707272745768, 0.3333333333333333703, 0.3249759707272745768, 0.3333333333333333703, 0.3249759707272745768, 0.3333333333333333703, 0.3249759707272745768, 0.3333333333333333703, 0.3249759707272745768, 0.3333333333333333703, 0.3249759707272745768, 0.3333333333333333703, 0.3249759707272745768, 0.3333333333333333703, 0.3249759707272745768, 0.3333333333333333703, 0.3249759707272745768, 0.3333333333333333703, 0.3249759707272745768, 0.3333333333333333703, 0.3249759707272745768, 0.3333333333333333703, 0.3249759707272745768, 0.3333333333333333703, 0.3249759707272745768, 0.3333333333333333703, 0.3249759707272745768, 0.3333333333333333703, 0.3249759707272745768, 0.3333333333333333703, 0.3249759707272745768, 0.3333333333333333703, 0.3249759707272745768, 0.3333333333333333703, 0.3249759707272745768, 0.3333333333333333703, 0.3249759707272745768, 0.3333333333333333703, 0.3249759707272745768, 0.3333333333333333703, 0.3249759707272745768, 0.3333333333333333703, 0.3249759707272745768, 0.3333333333333333703, 0.3249759707272745768, 0.3333333333333333703, 0.3249759707272745768, 0.3333333333333333703, 0.3249759707272745768, 0.3333333333333333703, 0.3249759707272745768, 0.3333333333333333703, 0.3249759707272745768, 0.3333333333333333703, 0.3249759707272745768, 0.3333333333333333703, 0.3291546520303039181, 0.3291546520303039736),
 ( 0.3333333333333333703, 0.3333333333333333703, 0.3333333333333333703, 0.3249759707272745768, 0.3333333333333333703, 0.3249759707272745768, 0.3333333333333333703, 0.3249759707272745768, 0.3333333333333333703, 0.3249759707272745768, 0.3333333333333333703, 0.3249759707272745768, 0.3333333333333333703, 0.3249759707272745768, 0.3333333333333333703, 0.3249759707272745768, 0.3333333333333333703, 0.3249759707272745768, 0.3333333333333333703, 0.3249759707272745768, 0.3333333333333333703, 0.3249759707272745768, 0.3333333333333333703, 0.3249759707272745768, 0.3333333333333333703, 0.3249759707272745768, 0.3333333333333333703, 0.3249759707272745768, 0.3333333333333333703, 0.3249759707272745768, 0.3333333333333333703, 0.3249759707272745768, 0.3333333333333333703, 0.3249759707272745768, 0.3333333333333333703, 0.3249759707272745768, 0.3333333333333333703, 0.3249759707272745768, 0.3333333333333333703, 0.3249759707272745768, 0.3333333333333333703, 0.3249759707272745768, 0.3333333333333333703, 0.3249759707272745768, 0.3333333333333333703, 0.3249759707272745768, 0.3333333333333333703, 0.3249759707272745768, 0.3333333333333333703, 0.3249759707272745768, 0.3333333333333333703, 0.3249759707272745768, 0.3333333333333333703, 0.3249759707272745768, 0.3333333333333333703, 0.3249759707272745768, 0.3333333333333333703, 0.3249759707272745768, 0.3333333333333333703, 0.3249759707272745768, 0.3333333333333333703, 0.3249759707272745768, 0.3333333333333333703, 0.3249759707272745768, 0.3333333333333333703, 0.3249759707272745768, 0.3333333333333333703, 0.3249759707272745768, 0.3333333333333333703, 0.3249759707272745768, 0.3333333333333333703, 0.3249759707272745768, 0.3333333333333333703, 0.3249759707272745768, 0.3333333333333333703, 0.3249759707272745768, 0.3333333333333333703, 0.3249759707272745768, 0.3333333333333333703, 0.3249759707272745768, 0.3333333333333333703, 0.3249759707272745768, 0.3333333333333333703, 0.3249759707272745768, 0.3333333333333333703, 0.3249759707272745768, 0.3333333333333333703, 0.3249759707272745768, 0.3333333333333333703, 0.3249759707272745768, 0.3333333333333333703, 0.3249759707272745768, 0.3333333333333333703, 0.3249759707272745768, 0.3333333333333333703, 0.3249759707272745768, 0.3333333333333333703, 0.3249759707272745768, 0.3333333333333333703, 0.3249759707272745768, 0.3333333333333333703, 0.3249759707272745768, 0.3333333333333333703, 0.3249759707272745768, 0.3333333333333333703, 0.3249759707272745768, 0.3333333333333333703, 0.3249759707272745768, 0.3333333333333333703, 0.3249759707272745768, 0.3333333333333333703, 0.3249759707272745768, 0.3333333333333333703, 0.3249759707272745768, 0.3333333333333333703, 0.3249759707272745768, 0.3333333333333333703, 0.3249759707272745768, 0.3333333333333333703, 0.3249759707272745768, 0.3333333333333333703, 0.3291546520303039181, 0.3291546520303039736),
 ( 1.000000000000000000, 1.000000000000000000, 1.000000000000000000, 0.9749279121818236193, 1.000000000000000000, 0.9749279121818236193, 1.000000000000000000, 0.9749279121818236193, 1.000000000000000000, 0.9749279121818236193, 1.000000000000000000, 0.9749279121818236193, 1.000000000000000000, 0.9749279121818236193, 1.000000000000000000, 0.9749279121818236193, 1.000000000000000000, 0.9749279121818236193, 1.000000000000000000, 0.9749279121818236193, 1.000000000000000000, 0.9749279121818236193, 1.000000000000000000, 0.9749279121818236193, 1.000000000000000000, 0.9749279121818236193, 1.000000000000000000, 0.9749279121818236193, 1.000000000000000000, 0.9749279121818236193, 1.000000000000000000, 0.9749279121818236193, 1.000000000000000000, 0.9749279121818236193, 1.000000000000000000, 0.9749279121818236193, 1.000000000000000000, 0.9749279121818236193, 1.000000000000000000, 0.9749279121818236193, 1.000000000000000000, 0.9749279121818236193, 1.000000000000000000, 0.9749279121818236193, 1.000000000000000000, 0.9749279121818236193, 1.000000000000000000, 0.9749279121818236193, 1.000000000000000000, 0.9749279121818236193, 1.000000000000000000, 0.9749279121818236193, 1.000000000000000000, 0.9749279121818236193, 1.000000000000000000, 0.9749279121818236193, 1.000000000000000000, 0.9749279121818236193, 1.000000000000000000, 0.9749279121818236193, 1.000000000000000000, 0.9749279121818236193, 1.000000000000000000, 0.9749279121818236193, 1.000000000000000000, 0.9749279121818236193, 1.000000000000000000, 0.9749279121818236193, 1.000000000000000000, 0.9749279121818236193, 1.000000000000000000, 0.9749279121818236193, 1.000000000000000000, 0.9749279121818236193, 1.000000000000000000, 0.9749279121818236193, 1.000000000000000000, 0.9749279121818236193, 1.000000000000000000, 0.9749279121818236193, 1.000000000000000000, 0.9749279121818236193, 1.000000000000000000, 0.9749279121818236193, 1.000000000000000000, 0.9749279121818236193, 1.000000000000000000, 0.9749279121818236193, 1.000000000000000000, 0.9749279121818236193, 1.000000000000000000, 0.9749279121818236193, 1.000000000000000000, 0.9749279121818236193, 1.000000000000000000, 0.9749279121818236193, 1.000000000000000000, 0.9749279121818236193, 1.000000000000000000, 0.9749279121818236193, 1.000000000000000000, 0.9749279121818236193, 1.000000000000000000, 0.9749279121818236193, 1.000000000000000000, 0.9749279121818236193, 1.000000000000000000, 0.9749279121818236193, 1.000000000000000000, 0.9749279121818236193, 1.000000000000000000, 0.9749279121818236193, 1.000000000000000000, 0.9749279121818236193, 1.000000000000000000, 0.9749279121818236193, 1.000000000000000000, 0.9749279121818236193, 1.000000000000000000, 0.9749279121818236193, 1.000000000000000000, 0.9874639560909115321, 0.9874639560909117542),
 ( 0.3333333333333333703, 0.3333333333333333703, 0.3333333333333333703, 0.3249759707272745768, 0.3333333333333333703, 0.3249759707272745768, 0.3333333333333333703, 0.3249759707272745768, 0.3333333333333333703, 0.3249759707272745768, 0.3333333333333333703, 0.3249759707272745768, 0.3333333333333333703, 0.3249759707272745768, 0.3333333333333333703, 0.3249759707272745768, 0.3333333333333333703, 0.3249759707272745768, 0.3333333333333333703, 0.3249759707272745768, 0.3333333333333333703, 0.3249759707272745768, 0.3333333333333333703, 0.3249759707272745768, 0.3333333333333333703, 0.3249759707272745768, 0.3333333333333333703, 0.3249759707272745768, 0.3333333333333333703, 0.3249759707272745768, 0.3333333333333333703, 0.3249759707272745768, 0.3333333333333333703, 0.3249759707272745768, 0.3333333333333333703, 0.3249759707272745768, 0.3333333333333333703, 0.3249759707272745768, 0.3333333333333333703, 0.3249759707272745768, 0.3333333333333333703, 0.3249759707272745768, 0.3333333333333333703, 0.3249759707272745768, 0.3333333333333333703, 0.3249759707272745768, 0.3333333333333333703, 0.3249759707272745768, 0.3333333333333333703, 0.3249759707272745768, 0.3333333333333333703, 0.3249759707272745768, 0.3333333333333333703, 0.3249759707272745768, 0.3333333333333333703, 0.3249759707272745768, 0.3333333333333333703, 0.3249759707272745768, 0.3333333333333333703, 0.3249759707272745768, 0.3333333333333333703, 0.3249759707272745768, 0.3333333333333333703, 0.3249759707272745768, 0.3333333333333333703, 0.3249759707272745768, 0.3333333333333333703, 0.3249759707272745768, 0.3333333333333333703, 0.3249759707272745768, 0.3333333333333333703, 0.3249759707272745768, 0.3333333333333333703, 0.3249759707272745768, 0.3333333333333333703, 0.3249759707272745768, 0.3333333333333333703, 0.3249759707272745768, 0.3333333333333333703, 0.3249759707272745768, 0.3333333333333333703, 0.3249759707272745768, 0.3333333333333333703, 0.3249759707272745768, 0.3333333333333333703, 0.3249759707272745768, 0.3333333333333333703, 0.3249759707272745768, 0.3333333333333333703, 0.3249759707272745768, 0.3333333333333333703, 0.3249759707272745768, 0.3333333333333333703, 0.3249759707272745768, 0.3333333333333333703, 0.3249759707272745768, 0.3333333333333333703, 0.3249759707272745768, 0.3333333333333333703, 0.3249759707272745768, 0.3333333333333333703, 0.3249759707272745768, 0.3333333333333333703, 0.3249759707272745768, 0.3333333333333333703, 0.3249759707272745768, 0.3333333333333333703, 0.3249759707272745768, 0.3333333333333333703, 0.3249759707272745768, 0.3333333333333333703, 0.3249759707272745768, 0.3333333333333333703, 0.3249759707272745768, 0.3333333333333333703, 0.3249759707272745768, 0.3333333333333333703, 0.3249759707272745768, 0.3333333333333333703, 0.3249759707272745768, 0.3333333333333333703, 0.3291546520303039181, 0.3291546520303039736),
 ( 0.3333333333333333703, 0.3333333333333333703, 0.3333333333333333703, 0.3249759707272745768, 0.3333333333333333703, 0.3249759707272745768, 0.3333333333333333703, 0.3249759707272745768, 0.3333333333333333703, 0.3249759707272745768, 0.3333333333333333703, 0.3249759707272745768, 0.3333333333333333703, 0.3249759707272745768, 0.3333333333333333703, 0.3249759707272745768, 0.3333333333333333703, 0.3249759707272745768, 0.3333333333333333703, 0.3249759707272745768, 0.3333333333333333703, 0.3249759707272745768, 0.3333333333333333703, 0.3249759707272745768, 0.3333333333333333703, 0.3249759707272745768, 0.3333333333333333703, 0.3249759707272745768, 0.3333333333333333703, 0.3249759707272745768, 0.3333333333333333703, 0.3249759707272745768, 0.3333333333333333703, 0.3249759707272745768, 0.3333333333333333703, 0.3249759707272745768, 0.3333333333333333703, 0.3249759707272745768, 0.3333333333333333703, 0.3249759707272745768, 0.3333333333333333703, 0.3249759707272745768, 0.3333333333333333703, 0.3249759707272745768, 0.3333333333333333703, 0.3249759707272745768, 0.3333333333333333703, 0.3249759707272745768, 0.3333333333333333703, 0.3249759707272745768, 0.3333333333333333703, 0.3249759707272745768, 0.3333333333333333703, 0.3249759707272745768, 0.3333333333333333703, 0.3249759707272745768, 0.3333333333333333703, 0.3249759707272745768, 0.3333333333333333703, 0.3249759707272745768, 0.3333333333333333703, 0.3249759707272745768, 0.3333333333333333703, 0.3249759707272745768, 0.3333333333333333703, 0.3249759707272745768, 0.3333333333333333703, 0.3249759707272745768, 0.3333333333333333703, 0.3249759707272745768, 0.3333333333333333703, 0.3249759707272745768, 0.3333333333333333703, 0.3249759707272745768, 0.3333333333333333703, 0.3249759707272745768, 0.3333333333333333703, 0.3249759707272745768, 0.3333333333333333703, 0.3249759707272745768, 0.3333333333333333703, 0.3249759707272745768, 0.3333333333333333703, 0.3249759707272745768, 0.3333333333333333703, 0.3249759707272745768, 0.3333333333333333703, 0.3249759707272745768, 0.3333333333333333703, 0.3249759707272745768, 0.3333333333333333703, 0.3249759707272745768, 0.3333333333333333703, 0.3249759707272745768, 0.3333333333333333703, 0.3249759707272745768, 0.3333333333333333703, 0.3249759707272745768, 0.3333333333333333703, 0.3249759707272745768, 0.3333333333333333703, 0.3249759707272745768, 0.3333333333333333703, 0.3249759707272745768, 0.3333333333333333703, 0.3249759707272745768, 0.3333333333333333703, 0.3249759707272745768, 0.3333333333333333703, 0.3249759707272745768, 0.3333333333333333703, 0.3249759707272745768, 0.3333333333333333703, 0.3249759707272745768, 0.3333333333333333703, 0.3249759707272745768, 0.3333333333333333703, 0.3249759707272745768, 0.3333333333333333703, 0.3249759707272745768, 0.3333333333333333703, 0.3291546520303039181, 0.3291546520303039736),
 ( 1.000000000000000000, 1.000000000000000000, 1.000000000000000000, 0.9749279121818236193, 1.000000000000000000, 0.9749279121818236193, 1.000000000000000000, 0.9749279121818236193, 1.000000000000000000, 0.9749279121818236193, 1.000000000000000000, 0.9749279121818236193, 1.000000000000000000, 0.9749279121818236193, 1.000000000000000000, 0.9749279121818236193, 1.000000000000000000, 0.9749279121818236193, 1.000000000000000000, 0.9749279121818236193, 1.000000000000000000, 0.9749279121818236193, 1.000000000000000000, 0.9749279121818236193, 1.000000000000000000, 0.9749279121818236193, 1.000000000000000000, 0.9749279121818236193, 1.000000000000000000, 0.9749279121818236193, 1.000000000000000000, 0.9749279121818236193, 1.000000000000000000, 0.9749279121818236193, 1.000000000000000000, 0.9749279121818236193, 1.000000000000000000, 0.9749279121818236193, 1.000000000000000000, 0.9749279121818236193, 1.000000000000000000, 0.9749279121818236193, 1.000000000000000000, 0.9749279121818236193, 1.000000000000000000, 0.9749279121818236193, 1.000000000000000000, 0.9749279121818236193, 1.000000000000000000, 0.9749279121818236193, 1.000000000000000000, 0.9749279121818236193, 1.000000000000000000, 0.9749279121818236193, 1.000000000000000000, 0.9749279121818236193, 1.000000000000000000, 0.9749279121818236193, 1.000000000000000000, 0.9749279121818236193, 1.000000000000000000, 0.9749279121818236193, 1.000000000000000000, 0.9749279121818236193, 1.000000000000000000, 0.9749279121818236193, 1.000000000000000000, 0.9749279121818236193, 1.000000000000000000, 0.9749279121818236193, 1.000000000000000000, 0.9749279121818236193, 1.000000000000000000, 0.9749279121818236193, 1.000000000000000000, 0.9749279121818236193, 1.000000000000000000, 0.9749279121818236193, 1.000000000000000000, 0.9749279121818236193, 1.000000000000000000, 0.9749279121818236193, 1.000000000000000000, 0.9749279121818236193, 1.000000000000000000, 0.9749279121818236193, 1.000000000000000000, 0.9749279121818236193, 1.000000000000000000, 0.9749279121818236193, 1.000000000000000000, 0.9749279121818236193, 1.000000000000000000, 0.9749279121818236193, 1.000000000000000000, 0.9749279121818236193, 1.000000000000000000, 0.9749279121818236193, 1.000000000000000000, 0.9749279121818236193, 1.000000000000000000, 0.9749279121818236193, 1.000000000000000000, 0.9749279121818236193, 1.000000000000000000, 0.9749279121818236193, 1.000000000000000000, 0.9749279121818236193, 1.000000000000000000, 0.9749279121818236193, 1.000000000000000000, 0.9749279121818236193, 1.000000000000000000, 0.9749279121818236193, 1.000000000000000000, 0.9749279121818236193, 1.000000000000000000, 0.9749279121818236193, 1.000000000000000000, 0.9749279121818236193, 1.000000000000000000, 0.9874639560909115321, 0.9874639560909117542) ) ) 
 REPRESENTATION_ITEM ( '' )  SURFACE ( )  );
#32520=CARTESIAN_POINT ( 'NONE',  ( 18.94344743393842379, -274.3916380513207969, -321.0982514603747973 ) ) ;
#32522=CARTESIAN_POINT ( 'NONE',  ( -38.92230237488710287, -288.9047901732640184, -347.3448935529162327 ) ) ;
#32524=CARTESIAN_POINT ( 'NONE',  ( 35.89035233665204316, -286.6199563678704862, -271.0502762912408343 ) ) ;
#32525=CARTESIAN_POINT ( 'NONE',  ( -105.4336747403305736, -288.9663577027548627, -238.7973145445781711 ) ) ;
#32527=CARTESIAN_POINT ( 'NONE',  ( 142.9247625494386114, 180.1091408837567371, -243.7470944784683127 ) ) ;
#32528=CARTESIAN_POINT ( 'NONE',  ( 21.21905379106112832, -287.6725291631148593, -314.0698889227368227 ) ) ;
#32530=CARTESIAN_POINT ( 'NONE',  ( -93.25192376431468233, -284.7730479017733956, -322.9814034909980478 ) ) ;
#32531=AXIS2_PLACEMENT_3D ( 'NONE', #19728, #91207, #69926 ) ;
#32532=CARTESIAN_POINT ( 'NONE',  ( -37.78161740844839755, -291.1055214671724229, -193.5976716885569715 ) ) ;
#32533=CARTESIAN_POINT ( 'NONE',  ( 19.51800930064586836, -282.4570673089704087, -219.6126778980658969 ) ) ;
#32534=CARTESIAN_POINT ( 'NONE',  ( 33.85928772399658016, -282.5084869852112774, -242.2216466203130665 ) ) ;
#32535=CARTESIAN_POINT ( 'NONE',  ( -69.01108493927020504, -283.3139436960800595, -336.1476363990104801 ) ) ;
#32536=CARTESIAN_POINT ( 'NONE',  ( 18.95283399503109933, -278.2412231387264114, -319.9378017746700493 ) ) ;
#32537=CARTESIAN_POINT ( 'NONE',  ( -101.5496900522852570, -297.1114765037191319, -227.8361201488905010 ) ) ;
#32538=CARTESIAN_POINT ( 'NONE',  ( -21.84627247365913050, -275.5700987234985178, -198.5200767987247161 ) ) ;
#32539=CARTESIAN_POINT ( 'NONE',  ( -1.630855336697323299, -290.5479465435475959, -204.7982798323102429 ) ) ;
#32541=CARTESIAN_POINT ( 'NONE',  ( -102.3751945454019108, -271.8089483051880961, -236.2249873332977188 ) ) ;
#32544=CARTESIAN_POINT ( 'NONE',  ( -108.3523298941789648, -286.1820054077951454, -292.6950531118995968 ) ) ;
#32545=CARTESIAN_POINT ( 'NONE',  ( -0.8411337741704904003, -295.6587920977971180, -337.8237109144015449 ) ) ;
#32546=CARTESIAN_POINT ( 'NONE',  ( -71.23283552471657742, -286.2436463648190283, -205.5901089585561010 ) ) ;
#32547=CARTESIAN_POINT ( 'NONE',  ( 38.90242257371527757, -274.7284465392191350, -279.7311097166445961 ) ) ;
#32548=CARTESIAN_POINT ( 'NONE',  ( 32.09035506203767341, -293.7779260142291378, -237.1843730163055000 ) ) ;
#32549=CARTESIAN_POINT ( 'NONE',  ( -13.07652042498867928, -284.5037083708650130, -198.5871217649060725 ) ) ;
#32550=CARTESIAN_POINT ( 'NONE',  ( -22.20210260406828695, -292.5741117308735397, -194.8314014930393512 ) ) ;
#32551=CARTESIAN_POINT ( 'NONE',  ( -42.66121851866647319, -289.4542498486399609, -343.2388620441287230 ) ) ;
#32554=CARTESIAN_POINT ( 'NONE',  ( 153.7037580466550821, 204.4818557570326902, -214.3672810361624954 ) ) ;
#32555=CARTESIAN_POINT ( 'NONE',  ( -43.62862356746156678, -287.4943387594404385, -194.2611003048058080 ) ) ;
#32556=CARTESIAN_POINT ( 'NONE',  ( -110.4683760289727132, -293.8380690714490129, -287.0191576251351080 ) ) ;
#32558=CARTESIAN_POINT ( 'NONE',  ( 19.58339992406645180, -281.1235365961811112, -316.5735305848129997 ) ) ;
#32559=CARTESIAN_POINT ( 'NONE',  ( -98.78910984784262439, -277.6009742027237621, -316.7504160945661056 ) ) ;
#32560=CARTESIAN_POINT ( 'NONE',  ( -88.80956642426248493, -281.3280777181398093, -215.9655722439982810 ) ) ;
#32561=CARTESIAN_POINT ( 'NONE',  ( 7.628150327998172386, -59.94677518897242408, -352.6193804921139758 ) ) ;
#32562=CARTESIAN_POINT ( 'NONE',  ( 23.77282892130728698, -280.7420612147766974, -316.2263622695442677 ) ) ;
#32563=CARTESIAN_POINT ( 'NONE',  ( 19.93982566509851395, -284.9077454862041918, -222.4802139764734363 ) ) ;
#32564=CARTESIAN_POINT ( 'NONE',  ( -93.25005675248959847, -275.1194957952901063, -219.2091760476533864 ) ) ;
#32565=CARTESIAN_POINT ( 'NONE',  ( -53.15659392583427945, -295.7526531643723615, -341.7425053747863899 ) ) ;
#32567=CARTESIAN_POINT ( 'NONE',  ( -4.598420262554686389, -291.1776227519213762, -204.5510410903042953 ) ) ;
#32568=CARTESIAN_POINT ( 'NONE',  ( 35.96796492082727070, -276.4957529148528579, -293.5776163616141048 ) ) ;
#32569=CARTESIAN_POINT ( 'NONE',  ( -56.86161410190220522, -273.7934600391721460, -199.9665721671149754 ) ) ;
#32570=CARTESIAN_POINT ( 'NONE',  ( 21.62204935220675495, -273.8102839982756791, -221.3226763461425151 ) ) ;
#32572=CARTESIAN_POINT ( 'NONE',  ( -98.10083840596374216, -271.1517187724923019, -226.3059262207511324 ) ) ;
#32573=CARTESIAN_POINT ( 'NONE',  ( -8.592757392746911194, -296.1085985611081810, -341.2133927272473670 ) ) ;
#32576=CARTESIAN_POINT ( 'NONE',  ( -107.6846607907899056, -285.3593448261918866, -291.0479521449954632 ) ) ;
#32577=CARTESIAN_POINT ( 'NONE',  ( 37.25555664430955716, -283.1289766948790998, -255.8965648295680637 ) ) ;
#32578=CARTESIAN_POINT ( 'NONE',  ( -101.8650957439092650, -283.4318674650633056, -304.8290872300131582 ) ) ;
#32579=CARTESIAN_POINT ( 'NONE',  ( -46.02220270507082489, -275.5637852912332733, -343.7000149732379555 ) ) ;
#32580=CARTESIAN_POINT ( 'NONE',  ( -64.48532464259463381, -285.2706934516060073, -339.4559016423420417 ) ) ;
#32581=CARTESIAN_POINT ( 'NONE',  ( -87.58222021782127342, -276.2489144919182991, -324.2739911415999359 ) ) ;
#32582=CARTESIAN_POINT ( 'NONE',  ( 32.35140462297783159, -276.3294134809819411, -247.4581411124910630 ) ) ;
#32584=CARTESIAN_POINT ( 'NONE',  ( -71.17272845035346052, -280.4197192067070432, -201.3711162142269586 ) ) ;
#32588=CARTESIAN_POINT ( 'NONE',  ( -35.20716411502890963, -287.9390621576985723, -194.6134557383130073 ) ) ;
#32589=CARTESIAN_POINT ( 'NONE',  ( -93.21231361429809681, -295.0793352926049806, -317.6147993215997190 ) ) ;
#32591=CARTESIAN_POINT ( 'NONE',  ( -113.0344426688517814, -289.7299764032954386, -283.9973048989509152 ) ) ;
#32592=CARTESIAN_POINT ( 'NONE',  ( -4.313967146831214627, -285.0710969631329590, -204.5998545141580109 ) ) ;
#32593=CARTESIAN_POINT ( 'NONE',  ( -82.32743018945153324, -289.6688381264211785, -211.5233428701100991 ) ) ;
#32594=CARTESIAN_POINT ( 'NONE',  ( -110.6257117043976592, -285.8216191337056671, -265.4538637725397621 ) ) ;
#32595=CARTESIAN_POINT ( 'NONE',  ( 25.94708344254813781, -274.0946431780135413, -310.7009957916968119 ) ) ;
#32596=CARTESIAN_POINT ( 'NONE',  ( 33.29301819966787690, -286.3203733230026842, -299.0878774437168204 ) ) ;
#32597=CARTESIAN_POINT ( 'NONE',  ( -21.43367214812339938, -288.2563288124215433, -197.0676306086918430 ) ) ;
#32598=CARTESIAN_POINT ( 'NONE',  ( 31.05466940947928478, -285.1423027177601170, -239.0593728467056849 ) ) ;
#32599=CARTESIAN_POINT ( 'NONE',  ( 20.37378398356347731, -283.1267792657722566, -315.4425037494083881 ) ) ;
#32600=CARTESIAN_POINT ( 'NONE',  ( -2.624290777631910210, -290.5942469099274490, -337.0299256629942306 ) ) ;
#32603=CARTESIAN_POINT ( 'NONE',  ( -100.4125407091589324, -297.9136228988910489, -312.0655920973689490 ) ) ;
#32605=CARTESIAN_POINT ( 'NONE',  ( -65.54522211681664601, -277.6832125674926601, -200.8660678185027280 ) ) ;
#32606=CARTESIAN_POINT ( 'NONE',  ( 17.38180141793691647, -292.0063132420249303, -216.3464293578725517 ) ) ;
#32607=CARTESIAN_POINT ( 'NONE',  ( -103.2375753620756740, -295.3995041303965081, -237.0182795954090125 ) ) ;
#32608=CARTESIAN_POINT ( 'NONE',  ( 24.10398729477568835, -279.6806568240900219, -229.9497019746799538 ) ) ;
#32609=CARTESIAN_POINT ( 'NONE',  ( -35.32732633982873693, -272.1574449580455735, -195.9356220532301620 ) ) ;
#32610=CARTESIAN_POINT ( 'NONE',  ( 26.22756049788171850, -295.3698947154877601, -307.2419067558803363 ) ) ;
#32611=CARTESIAN_POINT ( 'NONE',  ( -113.5916813653544324, -271.1988319013034356, -264.6520495995177953 ) ) ;
#32612=CARTESIAN_POINT ( 'NONE',  ( 37.81098343651878935, -291.9342970149134544, -281.5882354615037002 ) ) ;
#32613=CARTESIAN_POINT ( 'NONE',  ( -33.49564653083918131, -293.5267524977109019, -196.8598672718253511 ) ) ;
#32615=CARTESIAN_POINT ( 'NONE',  ( 35.06609209193271681, -294.2171184629137315, -259.8867037813033107 ) ) ;
#32617=CARTESIAN_POINT ( 'NONE',  ( -11.29474762352851691, -280.7346911788825423, -341.1269635043336734 ) ) ;
#32618=CARTESIAN_POINT ( 'NONE',  ( 25.79266356301712548, -294.0549325069128486, -307.0087935066652562 ) ) ;
#32619=CARTESIAN_POINT ( 'NONE',  ( -5.455519030079051035, -282.6441329965845171, -340.4487164218373891 ) ) ;
#32620=CARTESIAN_POINT ( 'NONE',  ( -112.5053660341964274, -284.0109811661047274, -286.9794096883084649 ) ) ;
#32621=CARTESIAN_POINT ( 'NONE',  ( -111.4418288685744187, -288.4163302953746779, -280.9031186873637012 ) ) ;
#32623=CARTESIAN_POINT ( 'NONE',  ( 38.49598568334300097, -279.9195783348995974, -261.4503271250531498 ) ) ;
#32624=CARTESIAN_POINT ( 'NONE',  ( -1.955624179986581668, -287.5149129998451940, -338.4002107134614903 ) ) ;
#32626=CARTESIAN_POINT ( 'NONE',  ( -17.99133341322022872, -296.3986251899053173, -341.5791193670521579 ) ) ;
#32627=CARTESIAN_POINT ( 'NONE',  ( 23.90631692584607748, -277.5898391021814291, -316.0479508920313378 ) ) ;
#32628=CARTESIAN_POINT ( 'NONE',  ( -70.94762243691920389, -279.2626800250376391, -205.5185648521822657 ) ) ;
#32629=CARTESIAN_POINT ( 'NONE',  ( 20.37728320186107567, -293.0284912539166839, -219.3753376206050518 ) ) ;
#32630=CARTESIAN_POINT ( 'NONE',  ( -105.3718039394970845, -283.0619493256399437, -237.4792206750342132 ) ) ;
#32631=CARTESIAN_POINT ( 'NONE',  ( -38.48816034180434542, -279.0666862744751029, -345.3523593491173642 ) ) ;
#32632=CARTESIAN_POINT ( 'NONE',  ( -5.929873331001648928, -291.5342566468563064, -204.1906158462052474 ) ) ;
#32633=CARTESIAN_POINT ( 'NONE',  ( -95.77176462076158714, -295.1990049728523218, -223.3406095111847947 ) ) ;
#32636=CARTESIAN_POINT ( 'NONE',  ( -3.120477932512370156, -294.0947776773638225, -334.9126198492454023 ) ) ;
#32637=CARTESIAN_POINT ( 'NONE',  ( 133.0380396672494783, -299.5541904835127980, -201.5129295623840449 ) ) ;
#32638=CARTESIAN_POINT ( 'NONE',  ( 30.89617123739170168, -285.2666405000203440, -285.9686137636504668 ) ) ;
#32639=CARTESIAN_POINT ( 'NONE',  ( -97.67990044980372488, -272.3869977470603772, -222.7852795422845986 ) ) ;
#32640=CARTESIAN_POINT ( 'NONE',  ( 38.04650232677378341, -279.7940556838514112, -278.4112173359901021 ) ) ;
#32643=CARTESIAN_POINT ( 'NONE',  ( -70.86534981146397172, -286.9342654913240267, -201.5900253128242241 ) ) ;
#32644=CARTESIAN_POINT ( 'NONE',  ( 16.00951215050787368, -288.1027900811589575, -320.2612584891847405 ) ) ;
#32645=CARTESIAN_POINT ( 'NONE',  ( -105.9058627385197724, -279.7144267401990874, -297.3733995713358809 ) ) ;
#32646=CARTESIAN_POINT ( 'NONE',  ( -70.94740970461043617, -299.3626559870327810, -204.4028662670947938 ) ) ;
#32647=CARTESIAN_POINT ( 'NONE',  ( -51.37173314567550619, -276.0304839186034656, -342.4047761157377749 ) ) ;
#32649=CARTESIAN_POINT ( 'NONE',  ( -37.24935154739976895, -297.7200014266754806, -193.3815033725163914 ) ) ;
#32650=CARTESIAN_POINT ( 'NONE',  ( -111.0453187876244243, -292.3360123529516841, -280.8970101591545472 ) ) ;
#32651=CARTESIAN_POINT ( 'NONE',  ( 23.32580779890089673, -294.5311298411430698, -224.2322362664154412 ) ) ;
#32652=CARTESIAN_POINT ( 'NONE',  ( -114.0438498160389287, -273.6021560138187851, -270.3744733279939965 ) ) ;
#32653=CARTESIAN_POINT ( 'NONE',  ( -78.22456173008137625, -290.2692494534612138, -331.0230789929115645 ) ) ;
#32655=CARTESIAN_POINT ( 'NONE',  ( -6.369840509506259352, -290.5942145151285558, -201.2019235178256338 ) ) ;
#32656=CARTESIAN_POINT ( 'NONE',  ( -80.61664344311897423, -297.8163796204223672, -206.6336646993826207 ) ) ;
#32657=CARTESIAN_POINT ( 'NONE',  ( -60.51858921352709331, -297.4099558805892798, -201.0622787149973760 ) ) ;
#32660=CARTESIAN_POINT ( 'NONE',  ( -93.07305233325782012, -291.3542938526953208, -322.5594508509145157 ) ) ;
#32661=CARTESIAN_POINT ( 'NONE',  ( 40.64545035920995986, -295.8376638359844719, -252.5284128619064461 ) ) ;
#32662=CARTESIAN_POINT ( 'NONE',  ( -96.41971609698404677, -287.1838143107498809, -224.4075638634668621 ) ) ;
#32663=CARTESIAN_POINT ( 'NONE',  ( -43.61094082968497787, -271.9727322639777753, -195.7388650299787685 ) ) ;
#32664=CARTESIAN_POINT ( 'NONE',  ( -66.39732374049609120, -275.5888570046891459, -201.8258355646289601 ) ) ;
#32665=CARTESIAN_POINT ( 'NONE',  ( -37.52951084827729034, -290.1296663984609836, -195.9086612669253213 ) ) ;
#32666=CARTESIAN_POINT ( 'NONE',  ( -110.2454055409880027, -280.1498624873998438, -290.9852596366845319 ) ) ;
#32667=AXIS2_PLACEMENT_3D ( 'NONE', #37757, #8426, #1327 ) ;
#32669=CARTESIAN_POINT ( 'NONE',  ( 13.99036024220834307, -281.6572649159380148, -322.4795930979910850 ) ) ;
#32670=CARTESIAN_POINT ( 'NONE',  ( -112.7591302074039845, -279.4561518100393300, -284.3509493984951177 ) ) ;
#32671=CARTESIAN_POINT ( 'NONE',  ( -19.83199417319972468, -279.0671977339699197, -195.7317056704644642 ) ) ;
#32672=CARTESIAN_POINT ( 'NONE',  ( 151.8863250319597000, 206.1547615615816369, -215.0904922897478571 ) ) ;
#32673=CARTESIAN_POINT ( 'NONE',  ( 24.18627271408411517, -277.1058970528413852, -316.2645903081284473 ) ) ;
#32674=CARTESIAN_POINT ( 'NONE',  ( -60.67766905526730170, -275.2750443224867354, -197.6551726798747666 ) ) ;
#32675=CARTESIAN_POINT ( 'NONE',  ( -69.91165696735023971, -300.1233781216987495, -202.8022627189028810 ) ) ;
#32677=VERTEX_POINT ( 'NONE', #23261 ) ;
#32678=CARTESIAN_POINT ( 'NONE',  ( 115.2940338803257703, -299.5541904835127980, -195.3611179825600175 ) ) ;
#32679=CARTESIAN_POINT ( 'NONE',  ( -39.95528097930107236, -290.1653046653184447, -343.6734138299510164 ) ) ;
#32680=CARTESIAN_POINT ( 'NONE',  ( 15.57720452528313615, -288.5486078092118305, -215.8307269825707806 ) ) ;
#32681=CARTESIAN_POINT ( 'NONE',  ( -78.23830235994276450, -288.9666328197043867, -331.0138154508651951 ) ) ;
#32682=CARTESIAN_POINT ( 'NONE',  ( 12.04288400302199236, -286.2249774361969799, -211.2942224539150118 ) ) ;
#32684=CARTESIAN_POINT ( 'NONE',  ( 34.71717841895296885, -280.1599667270440932, -286.2971915320982248 ) ) ;
#32685=CARTESIAN_POINT ( 'NONE',  ( 31.09138531498125957, -289.0313554288577507, -241.4569604033299015 ) ) ;
#32686=CARTESIAN_POINT ( 'NONE',  ( -74.15982291388664294, -282.0304562259884165, -334.2560491917651007 ) ) ;
#32687=CARTESIAN_POINT ( 'NONE',  ( -108.0976141132162383, -280.1287721598358758, -250.4437513797489601 ) ) ;
#32688=CARTESIAN_POINT ( 'NONE',  ( 39.11417577550911773, -288.5796958911892034, -277.2400170453149144 ) ) ;
#32689=CARTESIAN_POINT ( 'NONE',  ( -72.86644624274327953, -278.0286605184971336, -334.2189201317901848 ) ) ;
#32690=CARTESIAN_POINT ( 'NONE',  ( -113.8554361869827147, -289.3006209270952809, -274.0566439086643982 ) ) ;
#32691=CARTESIAN_POINT ( 'NONE',  ( -101.2790848122431697, -284.7918001381394788, -313.0731113635339966 ) ) ;
#32692=CARTESIAN_POINT ( 'NONE',  ( -10.02168170507467870, -286.8916785981275552, -198.3797964384549743 ) ) ;
#32693=CARTESIAN_POINT ( 'NONE',  ( -58.94610623450461162, -283.5061290872394011, -340.1440924515371762 ) ) ;
#32696=CARTESIAN_POINT ( 'NONE',  ( -111.9132769292164227, -292.2413997197231765, -283.8277560848690655 ) ) ;
#32697=CARTESIAN_POINT ( 'NONE',  ( 19.15413177870801320, -292.9436305070307753, -322.0281775360701886 ) ) ;
#32698=CARTESIAN_POINT ( 'NONE',  ( 33.46663503010690022, -274.8569971919787918, -289.0583937417505922 ) ) ;
#32699=CARTESIAN_POINT ( 'NONE',  ( -110.2517025824968471, -295.5925449256187107, -294.8037923163639107 ) ) ;
#32700=CARTESIAN_POINT ( 'NONE',  ( -22.58303012936103826, -290.7243881366661640, -198.1607758059705020 ) ) ;
#32701=CARTESIAN_POINT ( 'NONE',  ( -23.34892642947344399, -293.1107942557617889, -343.0920182071574231 ) ) ;
#32702=CARTESIAN_POINT ( 'NONE',  ( -110.6431755441068532, -291.8180519338893077, -265.7257515580950553 ) ) ;
#32704=CARTESIAN_POINT ( 'NONE',  ( 36.52837220358623682, -291.3739008384073941, -256.4600085735470429 ) ) ;
#32705=CARTESIAN_POINT ( 'NONE',  ( 31.16687527362607923, -295.9537693457886576, -301.0088487393136916 ) ) ;
#32706=CARTESIAN_POINT ( 'NONE',  ( 34.99350743265259212, -288.6449753292862965, -281.8877846085155170 ) ) ;
#32707=CARTESIAN_POINT ( 'NONE',  ( 19.59440823066776005, -278.2137872534224812, -319.7434591597016151 ) ) ;
#32708=CARTESIAN_POINT ( 'NONE',  ( -56.83786395635641497, -276.0929264183029090, -344.4963078425350318 ) ) ;
#32710=CARTESIAN_POINT ( 'NONE',  ( -91.51442520256379964, -296.5014636604155385, -215.8682314903987276 ) ) ;
#32711=CARTESIAN_POINT ( 'NONE',  ( 18.18075961690786713, -274.4815289224268895, -319.3213225810429776 ) ) ;
#32712=CARTESIAN_POINT ( 'NONE',  ( -19.15962067499798849, -278.3676429771831522, -198.1224316850475589 ) ) ;
#32713=CARTESIAN_POINT ( 'NONE',  ( 33.97598714308885803, -276.9854976929820509, -287.7610961014028135 ) ) ;
#32714=CARTESIAN_POINT ( 'NONE',  ( -42.76973140434803611, -275.5194496314200023, -346.3675446327143277 ) ) ;
#32716=CARTESIAN_POINT ( 'NONE',  ( -33.81255125181687760, -298.9002774137236997, -197.1991438378180703 ) ) ;
#32718=CARTESIAN_POINT ( 'NONE',  ( 9.192011959814715638, -286.4372534842286768, -329.6982213110718476 ) ) ;
#32719=CARTESIAN_POINT ( 'NONE',  ( -31.33759439226609800, -273.9633785012337626, -197.5958002610799156 ) ) ;
#32720=CARTESIAN_POINT ( 'NONE',  ( 35.84903297082797735, -287.2492998703770581, -246.2716405601228189 ) ) ;
#32721=CARTESIAN_POINT ( 'NONE',  ( -45.96717373674685803, -299.9231724059632143, -195.5011954164149870 ) ) ;
#32722=CARTESIAN_POINT ( 'NONE',  ( -94.11917273739189227, -295.2291774508144613, -221.5936262951379661 ) ) ;
#32723=CARTESIAN_POINT ( 'NONE',  ( 6.101395986104649616, -279.8226124486786830, -206.9824447548156172 ) ) ;
#32725=CARTESIAN_POINT ( 'NONE',  ( -10.41089955328140881, -278.4032439015824139, -200.3082946097797787 ) ) ;
#32727=CARTESIAN_POINT ( 'NONE',  ( -109.0539615864481959, -289.1412154093627578, -286.0555242936515015 ) ) ;
#32729=CARTESIAN_POINT ( 'NONE',  ( -68.61247857462009847, -289.6410736226715130, -202.1770821698003431 ) ) ;
#32730=CARTESIAN_POINT ( 'NONE',  ( -57.06563122903368424, -275.3133373570557296, -199.3031485292505920 ) ) ;
#32731=CARTESIAN_POINT ( 'NONE',  ( -27.43040745016602244, -284.3539821233872544, -346.1793180783183175 ) ) ;
#32732=CARTESIAN_POINT ( 'NONE',  ( -98.38890591690906717, -271.2352666404831325, -225.7485269746892982 ) ) ;
#32733=CARTESIAN_POINT ( 'NONE',  ( -63.53326811574574862, -275.1292870704504594, -201.5770503216591294 ) ) ;
#32734=CARTESIAN_POINT ( 'NONE',  ( -36.74500083477536805, -274.8626726804567397, -197.1896319917300389 ) ) ;
#32735=CARTESIAN_POINT ( 'NONE',  ( -16.66803297545346751, -284.7853767115535675, -342.5093573545170216 ) ) ;
#32736=CARTESIAN_POINT ( 'NONE',  ( -87.53497357235173126, -272.2523024649440231, -216.8607253488772528 ) ) ;
#32738=CARTESIAN_POINT ( 'NONE',  ( 204.2025551593094121, 295.5631162206468048, -54.00000000005014300 ) ) ;
#32739=CARTESIAN_POINT ( 'NONE',  ( 37.09602283697132208, -293.6320802033485506, -290.0594784296054627 ) ) ;
#32740=CARTESIAN_POINT ( 'NONE',  ( -108.9396684218322804, -286.8072870316539706, -249.0729263399446722 ) ) ;
#32742=CARTESIAN_POINT ( 'NONE',  ( 40.64545035920995986, -273.2666405000204009, -288.1938231032136741 ) ) ;
#32743=CARTESIAN_POINT ( 'NONE',  ( -109.5884415500002831, -277.4164148835582751, -296.6810596739367725 ) ) ;
#32745=CARTESIAN_POINT ( 'NONE',  ( -113.5680287832200719, -288.9773741573943084, -268.3552243968866264 ) ) ;
#32746=CARTESIAN_POINT ( 'NONE',  ( -0.8923988824507324003, -284.0788635948879346, -334.4091951720478164 ) ) ;
#32747=CARTESIAN_POINT ( 'NONE',  ( -29.58524501423735131, -278.7128792920361207, -344.0185153731196692 ) ) ;
#32748=CARTESIAN_POINT ( 'NONE',  ( -95.38098671520711491, -286.6538465493970875, -220.5821669827580251 ) ) ;
#32749=CARTESIAN_POINT ( 'NONE',  ( 20.35890362660326502, -282.8906745624727819, -222.4283470015218427 ) ) ;
#32750=CARTESIAN_POINT ( 'NONE',  ( 4.861386396898944362, -274.7716542881061628, -205.8936689348984146 ) ) ;
#32751=CARTESIAN_POINT ( 'NONE',  ( -87.09681114658178558, -277.5560523220985374, -329.1967657142477606 ) ) ;
#32752=CARTESIAN_POINT ( 'NONE',  ( -83.22861867451176465, -297.6059734263096743, -329.0417079162932623 ) ) ;
#32755=CARTESIAN_POINT ( 'NONE',  ( -35.83451943785929927, -296.2104197581550693, -194.5967821684023704 ) ) ;
#32756=CARTESIAN_POINT ( 'NONE',  ( -110.4535370110471462, -278.0562309456329899, -270.6320298648365110 ) ) ;
#32757=CARTESIAN_POINT ( 'NONE',  ( -49.67053651609517573, -275.1034798830269779, -194.7032998507759203 ) ) ;
#32758=CARTESIAN_POINT ( 'NONE',  ( 17.62840567704764183, -288.6121324885496620, -220.7815193943803536 ) ) ;
#32759=CARTESIAN_POINT ( 'NONE',  ( -103.9878321598168327, -297.5848638617578104, -307.6309074458534951 ) ) ;
#32760=CARTESIAN_POINT ( 'NONE',  ( -34.85209762121945687, -296.2265970318481436, -346.9235800576190627 ) ) ;
#32761=CARTESIAN_POINT ( 'NONE',  ( -95.73714348387795781, -293.1976446500661382, -223.5433050743689591 ) ) ;
#32762=CARTESIAN_POINT ( 'NONE',  ( -82.37124065772339065, -277.4361608060952449, -210.5267691309406359 ) ) ;
#32763=CARTESIAN_POINT ( 'NONE',  ( 30.27056421462915026, -283.0588207185207352, -239.0945237478530316 ) ) ;
#32764=CARTESIAN_POINT ( 'NONE',  ( -41.93320808914626951, -296.0736790091700641, -196.0628525008749534 ) ) ;
#32765=CARTESIAN_POINT ( 'NONE',  ( -38.68648037173607435, -284.9292604148132568, -346.1139862449836642 ) ) ;
#32766=CARTESIAN_POINT ( 'NONE',  ( 35.75898745660029476, -286.5533904706117028, -276.5209368664935710 ) ) ;
#32767=CARTESIAN_POINT ( 'NONE',  ( -110.3273273839884610, -271.8591574644645448, -296.2092911942687010 ) ) ;
#32769=CARTESIAN_POINT ( 'NONE',  ( -17.16196182006822113, -285.9865137319845303, -200.1308670104079397 ) ) ;
#32771=CARTESIAN_POINT ( 'NONE',  ( -38.71317819491038392, -284.1486422036933845, -347.0397431585845993 ) ) ;
#32772=CARTESIAN_POINT ( 'NONE',  ( -109.9072526409043036, -272.9928396826201720, -262.2169129720123806 ) ) ;
#32773=CARTESIAN_POINT ( 'NONE',  ( 33.49811567641476984, -285.9731660756377210, -241.0723588670986999 ) ) ;
#32774=CARTESIAN_POINT ( 'NONE',  ( 18.97935819681732639, -281.7806702549289071, -218.2002264816921411 ) ) ;
#32776=CARTESIAN_POINT ( 'NONE',  ( -111.4175745230541850, -280.3040947252583805, -251.9915418739947484 ) ) ;
#32777=CARTESIAN_POINT ( 'NONE',  ( 32.00057492710987361, -281.4550965857262099, -236.8110679369113996 ) ) ;
#32778=CARTESIAN_POINT ( 'NONE',  ( -37.30987171927208834, -283.5523547857346784, -200.3611179825600459 ) ) ;
#32779=CARTESIAN_POINT ( 'NONE',  ( 85.34974711902751210, 82.93338734745742613, -302.3957557721062699 ) ) ;
#32781=CARTESIAN_POINT ( 'NONE',  ( 37.41704493807935705, -277.4962935497120498, -266.0075450164081303 ) ) ;
#32782=CARTESIAN_POINT ( 'NONE',  ( -78.55901433422972957, -208.1269654894091161, -356.8488242329224818 ) ) ;
#32783=CARTESIAN_POINT ( 'NONE',  ( 19.73613809064724833, -280.2407817075410890, -318.4846638550416174 ) ) ;
#32784=CARTESIAN_POINT ( 'NONE',  ( 19.60421918333060987, -294.6216950314292262, -220.0310675260219284 ) ) ;
#32785=CARTESIAN_POINT ( 'NONE',  ( -109.4648368559871017, -295.7436780642699432, -282.2836100399914585 ) ) ;
#32786=CARTESIAN_POINT ( 'NONE',  ( -2.078451881527334510, -292.0139868680623181, -201.9648466246572127 ) ) ;
#32788=CARTESIAN_POINT ( 'NONE',  ( -99.53953502503475192, -294.5334267876225454, -314.8353484836579810 ) ) ;
#32789=CARTESIAN_POINT ( 'NONE',  ( 35.35903407656502395, -285.7826613046892135, -257.3821092042276746 ) ) ;
#32790=CARTESIAN_POINT ( 'NONE',  ( 33.94281058225051595, -295.6826424963398381, -291.1284417734622139 ) ) ;
#32791=CARTESIAN_POINT ( 'NONE',  ( -107.0051002545059333, -286.1781570310841403, -246.7868294666612883 ) ) ;
#32792=CARTESIAN_POINT ( 'NONE',  ( 23.78058699239112173, -293.8723600156076259, -223.8972019567250413 ) ) ;
#32793=CARTESIAN_POINT ( 'NONE',  ( -109.5582071353410356, -284.8941864146328840, -281.7654377168906308 ) ) ;
#32794=CARTESIAN_POINT ( 'NONE',  ( -69.37592593356716009, -294.2592907575341883, -339.9586450198791567 ) ) ;
#32795=CARTESIAN_POINT ( 'NONE',  ( -112.9725432089030335, -291.1839872414853971, -284.0049950115785578 ) ) ;
#32796=CARTESIAN_POINT ( 'NONE',  ( -90.74773663520244327, -291.8118055955172281, -214.9037604585546148 ) ) ;
#32797=CARTESIAN_POINT ( 'NONE',  ( -73.54311925351944979, -289.7135556041953350, -333.7668319371736629 ) ) ;
#32800=CARTESIAN_POINT ( 'NONE',  ( -33.43809796967462944, -299.9609350218637474, -194.5950889648607358 ) ) ;
#32801=CARTESIAN_POINT ( 'NONE',  ( -21.42225531884626477, -273.0468653608984368, -195.4306168869844953 ) ) ;
#32802=CARTESIAN_POINT ( 'NONE',  ( 7.295195307877241575, -279.7361149232996809, -212.2370119380635458 ) ) ;
#32803=CARTESIAN_POINT ( 'NONE',  ( 18.04965236476250112, -274.3274023508747064, -216.8868334919154677 ) ) ;
#32804=CARTESIAN_POINT ( 'NONE',  ( -77.87734818954048421, -295.9769508176643171, -208.7565794703882318 ) ) ;
#32805=CARTESIAN_POINT ( 'NONE',  ( -83.76098006036900756, -279.5571295005846082, -328.3592544500821759 ) ) ;
#32806=CARTESIAN_POINT ( 'NONE',  ( -1.099232556023643337, -272.6780476209133326, -205.5596091420736400 ) ) ;
#32807=CARTESIAN_POINT ( 'NONE',  ( -110.7811908363420059, -297.7424968122513178, -271.4844253147840618 ) ) ;
#32808=CARTESIAN_POINT ( 'NONE',  ( -109.4436631883412332, -297.4568765994258683, -283.6794746251381412 ) ) ;
#32810=CARTESIAN_POINT ( 'NONE',  ( -96.73573769918829157, -298.7987109146243370, -222.6244578587956369 ) ) ;
#32811=CARTESIAN_POINT ( 'NONE',  ( -15.45078558823529669, -296.3254154660327231, -195.2018851504046779 ) ) ;
#32812=CARTESIAN_POINT ( 'NONE',  ( 6.130207696522662175, -295.0962149306045035, -329.1956788084126515 ) ) ;
#32813=CARTESIAN_POINT ( 'NONE',  ( 21.47560178783512086, -291.5108351405484655, -226.1355607345328167 ) ) ;
#32815=CARTESIAN_POINT ( 'NONE',  ( 13.91880144552290766, -275.2406749740655982, -212.9149523058738396 ) ) ;
#32816=CARTESIAN_POINT ( 'NONE',  ( -33.81508741270545926, -298.4307796347532644, -197.3397675358135075 ) ) ;
#32817=CARTESIAN_POINT ( 'NONE',  ( -1.142926231357398237, -284.5542307995082751, -336.4670071600247070 ) ) ;
#32818=CARTESIAN_POINT ( 'NONE',  ( -55.60081723594127823, -281.9672368499194590, -344.6571670960450433 ) ) ;
#32819=CARTESIAN_POINT ( 'NONE',  ( 3.440400404170164794, -275.8681050273172559, -335.6168395218352316 ) ) ;
#32821=CARTESIAN_POINT ( 'NONE',  ( -56.37072695869962757, -282.5008803965488937, -341.0045739027429477 ) ) ;
#32822=CARTESIAN_POINT ( 'NONE',  ( 25.18243166846312775, -280.1146008824209162, -312.0835504337774751 ) ) ;
#32823=CARTESIAN_POINT ( 'NONE',  ( 35.20961297883029317, -273.9647282484440893, -257.9702451927489619 ) ) ;
#32824=CARTESIAN_POINT ( 'NONE',  ( -111.3020683139406373, -280.7130718518005210, -257.8408025537938784 ) ) ;
#32828=CARTESIAN_POINT ( 'NONE',  ( -63.26557735654754566, -272.1198406178012874, -198.7064391107515746 ) ) ;
#32829=CARTESIAN_POINT ( 'NONE',  ( -94.73252445600395788, -279.8821134031131237, -318.9229339386325250 ) ) ;
#32831=CARTESIAN_POINT ( 'NONE',  ( -110.4749258510289422, -286.2294267523125200, -289.4082818517500186 ) ) ;
#32834=CARTESIAN_POINT ( 'NONE',  ( -8.418478753352225397, -286.6733960011205227, -339.5734022241688308 ) ) ;
#32836=CARTESIAN_POINT ( 'NONE',  ( -84.74619556927338238, -294.5172605550152412, -326.4630669486883221 ) ) ;
#32837=CARTESIAN_POINT ( 'NONE',  ( -12.90321945535889725, -286.8707148162086469, -340.4583799957183032 ) ) ;
#32838=CARTESIAN_POINT ( 'NONE',  ( -107.8893720497363518, -252.3744610414916565, -325.2219058921743908 ) ) ;
#32839=CARTESIAN_POINT ( 'NONE',  ( -112.3745884092469964, -294.5737924874119358, -268.6628699735679788 ) ) ;
#32840=CARTESIAN_POINT ( 'NONE',  ( -36.55297794806401868, -284.5417667913201853, -194.0456032211958188 ) ) ;
#32841=CARTESIAN_POINT ( 'NONE',  ( -14.07578509605410666, -281.9590349963796712, -200.2704108289871954 ) ) ;
#32842=CARTESIAN_POINT ( 'NONE',  ( -100.5883263543587844, -282.2292397523884802, -312.5725292539780185 ) ) ;
#32843=CARTESIAN_POINT ( 'NONE',  ( 16.01096319219574582, -288.2694432291956446, -320.2597071249346641 ) ) ;
#32844=CARTESIAN_POINT ( 'NONE',  ( -93.55193220931684550, -280.6471505415067327, -222.8466261922679053 ) ) ;
#32845=CARTESIAN_POINT ( 'NONE',  ( 15.36863879043039560, -281.6233061980023535, -219.5519667075348593 ) ) ;
#32847=CARTESIAN_POINT ( 'NONE',  ( 4.661860201572728180, -290.4680066554457767, -332.9239481646301897 ) ) ;
#32849=CARTESIAN_POINT ( 'NONE',  ( -90.16285924102847105, -273.3302529751937868, -214.2621941111483181 ) ) ;
#32850=CARTESIAN_POINT ( 'NONE',  ( -110.2642716376925591, -292.3256672490841765, -286.3623808589996997 ) ) ;
#32851=DIRECTION ( 'NONE',  ( 0.000000000000000000, 0.000000000000000000, -1.000000000000000000 ) ) ;
#32852=CARTESIAN_POINT ( 'NONE',  ( -55.56934967048406548, -297.7662352645559167, -350.3683826091709648 ) ) ;
#32854=CARTESIAN_POINT ( 'NONE',  ( 21.19680668337102958, -274.1995948451560707, -317.5330495790701093 ) ) ;
#32856=CARTESIAN_POINT ( 'NONE',  ( -67.92400455736233766, -293.8468436901030145, -340.1548359867680915 ) ) ;
#32857=CARTESIAN_POINT ( 'NONE',  ( 5.242850644267413429, -273.9936478771248858, -210.8809696933471969 ) ) ;
#32858=CARTESIAN_POINT ( 'NONE',  ( 26.30453471381903441, -289.5785226112020609, -307.6085722133709623 ) ) ;
#32859=CARTESIAN_POINT ( 'NONE',  ( 18.38236746969534252, -283.9977485967817756, -319.0725366169236850 ) ) ;
#32860=CARTESIAN_POINT ( 'NONE',  ( -113.4219892818600783, -292.0737960958622352, -262.7141145182393984 ) ) ;
#32861=CARTESIAN_POINT ( 'NONE',  ( -81.65843981301547672, -292.7777780252258708, -207.9966661266957999 ) ) ;
#32862=CARTESIAN_POINT ( 'NONE',  ( -32.15516723932170606, -291.9526794001114354, -197.5329781575705965 ) ) ;
#32863=CARTESIAN_POINT ( 'NONE',  ( -102.7476271547374296, -287.0423280085199167, -233.5522329158753791 ) ) ;
#32864=CARTESIAN_POINT ( 'NONE',  ( 8.544836518185610075, -280.8276896247477907, -208.4609840811428114 ) ) ;
#32865=CARTESIAN_POINT ( 'NONE',  ( -93.59616042685664183, -293.9343861330013397, -320.8259167351917540 ) ) ;
#32866=CARTESIAN_POINT ( 'NONE',  ( -24.53567159286675903, -282.7264971892649896, -346.3428679147873481 ) ) ;
#32867=CARTESIAN_POINT ( 'NONE',  ( 35.32566966056675284, -277.2148960827357769, -255.1228946097576795 ) ) ;
#32869=CARTESIAN_POINT ( 'NONE',  ( 27.36219212280431989, -290.4805209788416391, -301.4846348637938149 ) ) ;
#32870=CARTESIAN_POINT ( 'NONE',  ( -23.19317750634681730, -275.0127936719401873, -344.8464457043886000 ) ) ;
#32872=CARTESIAN_POINT ( 'NONE',  ( -70.24825271200126053, -283.0055782943686609, -335.6065984688368644 ) ) ;
#32873=CARTESIAN_POINT ( 'NONE',  ( -103.0787761271877230, -280.2738394017300720, -230.9305307229744244 ) ) ;
#32874=CARTESIAN_POINT ( 'NONE',  ( 33.81969193680325958, -286.9791436470911776, -299.2928649801286838 ) ) ;
#32875=CARTESIAN_POINT ( 'NONE',  ( -38.94164880246820104, -293.7919499286405198, -196.3650763302414930 ) ) ;
#32876=CARTESIAN_POINT ( 'NONE',  ( 38.75411320653979885, -277.0904747896923368, -265.4706009359164796 ) ) ;
#32877=CARTESIAN_POINT ( 'NONE',  ( 23.98247542316440573, -277.4797586216487275, -316.1065414365120319 ) ) ;
#32878=CARTESIAN_POINT ( 'NONE',  ( -106.2649104874848831, -278.0636821907446574, -294.5683552148326498 ) ) ;
#32879=CARTESIAN_POINT ( 'NONE',  ( -35.79291522040858808, -300.0717403666205882, -195.5272464029587240 ) ) ;
#32880=CARTESIAN_POINT ( 'NONE',  ( -63.17237257271649042, -283.7149093589713402, -200.0719348275429468 ) ) ;
#32881=CARTESIAN_POINT ( 'NONE',  ( -2.061745773593721243, -292.1730271632944209, -201.9280050367528645 ) ) ;
#32882=CARTESIAN_POINT ( 'NONE',  ( 28.22585110764876504, -289.6633859786339258, -309.1855515133631229 ) ) ;
#32883=CARTESIAN_POINT ( 'NONE',  ( 36.01723295166004135, -292.4779153790240116, -270.7753333347918669 ) ) ;
#32885=EDGE_CURVE ( 'NONE', #43403, #29794, #41418, .T. ) ;
#32886=CARTESIAN_POINT ( 'NONE',  ( -64.16482900053965466, -290.2838308103768554, -198.7573126711144198 ) ) ;
#32887=CARTESIAN_POINT ( 'NONE',  ( -9.715543979829012855, -292.0898342371773992, -202.7138029605008853 ) ) ;
#32889=CARTESIAN_POINT ( 'NONE',  ( -4.453108471476115326, -289.7085324850863799, -339.6563682527219044 ) ) ;
#32890=CARTESIAN_POINT ( 'NONE',  ( -95.63119207124971410, -279.5033083319034972, -226.3582899885431061 ) ) ;
#32891=CARTESIAN_POINT ( 'NONE',  ( -97.98106593156762756, -296.1020592677214154, -223.3893188395267657 ) ) ;
#32892=CARTESIAN_POINT ( 'NONE',  ( -46.50159475958982114, -286.5902049458972556, -194.0105507498423094 ) ) ;
#32893=CARTESIAN_POINT ( 'NONE',  ( -20.99259590879864845, -286.5897177621790206, -195.1384413307527552 ) ) ;
#32894=CARTESIAN_POINT ( 'NONE',  ( -78.38501105099166466, -283.9548810786728836, -330.7559365947181504 ) ) ;
#32895=CARTESIAN_POINT ( 'NONE',  ( -113.9562875489731653, -273.5685593820227837, -284.1604309951135861 ) ) ;
#32896=CARTESIAN_POINT ( 'NONE',  ( 152.1864817686872868, 207.0855559507159853, -216.2993369928966274 ) ) ;
#32897=CARTESIAN_POINT ( 'NONE',  ( 102.3144949715192240, 114.9274731801767331, -279.5273309297857054 ) ) ;
#32898=CARTESIAN_POINT ( 'NONE',  ( 5.279096791983114656, -273.8422528797663631, -210.8336381429203925 ) ) ;
#32899=CARTESIAN_POINT ( 'NONE',  ( 3.294073093163292665, -275.4120145335326129, -331.3771815049728389 ) ) ;
#32900=CARTESIAN_POINT ( 'NONE',  ( -105.1963761121639465, -296.5301306658017779, -233.9814681441946504 ) ) ;
#32901=CARTESIAN_POINT ( 'NONE',  ( 190.2888855011954945, 268.0502169937788040, -137.8993104347648284 ) ) ;
#32902=CARTESIAN_POINT ( 'NONE',  ( 38.43803421264869513, -274.1045306193429383, -259.8382792094398042 ) ) ;
#32903=CARTESIAN_POINT ( 'NONE',  ( -110.1303768051990346, -274.4903250376994492, -256.6782261879677662 ) ) ;
#32905=CARTESIAN_POINT ( 'NONE',  ( -94.86377098310568101, -274.3213539501816740, -219.6392895967927643 ) ) ;
#32906=CARTESIAN_POINT ( 'NONE',  ( -101.6943818429355133, -290.5718705282404812, -305.0620180383345428 ) ) ;
#32907=CARTESIAN_POINT ( 'NONE',  ( -81.76998556058332213, -296.4427856299671475, -333.1180936335334763 ) ) ;
#32908=CARTESIAN_POINT ( 'NONE',  ( -48.96688651821023797, -298.4003302111540279, -194.2523696570733023 ) ) ;
#32909=CARTESIAN_POINT ( 'NONE',  ( -53.14730905675413908, -295.4270384066023780, -341.6814875082871481 ) ) ;
#32910=EDGE_LOOP ( 'NONE', ( #8854, #17077, #40225, #31872 ) ) ;
#32911=CARTESIAN_POINT ( 'NONE',  ( -86.14609995477528059, -279.6425506022802097, -328.1135653219418487 ) ) ;
#32912=CARTESIAN_POINT ( 'NONE',  ( -39.57918236722738925, -279.5324500610237806, -193.4421573521956361 ) ) ;
#32913=CARTESIAN_POINT ( 'NONE',  ( 5.544245583410889466, -277.3968768583897599, -329.7887557370479499 ) ) ;
#32914=CARTESIAN_POINT ( 'NONE',  ( -4.413416606285027299, -278.3843189159451867, -338.8568285454893498 ) ) ;
#32915=CARTESIAN_POINT ( 'NONE',  ( -110.8848032877358918, -276.3623491326079602, -286.7872795933438965 ) ) ;
#32916=CARTESIAN_POINT ( 'NONE',  ( -68.31436617887244722, -274.1263777170876779, -204.1757949561956309 ) ) ;
#32917=CARTESIAN_POINT ( 'NONE',  ( -103.8223008511671992, -271.4580207823357227, -238.5643024504222467 ) ) ;
#32919=CARTESIAN_POINT ( 'NONE',  ( -110.3512522342016382, -278.7511626175920014, -267.9103805241133500 ) ) ;
#32920=CARTESIAN_POINT ( 'NONE',  ( 2.906367770195225742, -287.2091512239007329, -335.4877739259253531 ) ) ;
#32921=CARTESIAN_POINT ( 'NONE',  ( -82.39943295479227459, -275.4376479941607840, -210.3394393060066818 ) ) ;
#32923=CARTESIAN_POINT ( 'NONE',  ( -109.3396425958786864, -289.5782552270793531, -283.3571946096433862 ) ) ;
#32924=CARTESIAN_POINT ( 'NONE',  ( -105.6973469637469947, -283.4448292127206059, -305.7025755731332879 ) ) ;
#32925=CARTESIAN_POINT ( 'NONE',  ( 33.19024411569889565, -280.0873258821627019, -292.9604114228595790 ) ) ;
#32926=CARTESIAN_POINT ( 'NONE',  ( 19.30117814593473113, -279.4657959588715244, -223.3632693802757956 ) ) ;
#32927=CARTESIAN_POINT ( 'NONE',  ( -103.5073756568267527, -283.0867316973655647, -236.2522103950360020 ) ) ;
#32928=CARTESIAN_POINT ( 'NONE',  ( 36.94504401476538646, -289.6894933170121362, -281.0449711320229085 ) ) ;
#32929=CARTESIAN_POINT ( 'NONE',  ( -95.11285719183571530, -280.3922774516108234, -225.0681107466438675 ) ) ;
#32931=CARTESIAN_POINT ( 'NONE',  ( 17.92422182340621006, -294.8440684992285128, -219.6592588409577900 ) ) ;
#32932=CARTESIAN_POINT ( 'NONE',  ( -83.92776260473499406, -277.6624315775244440, -210.2636143687693959 ) ) ;
#32933=CARTESIAN_POINT ( 'NONE',  ( 17.51721007319650525, -276.8926937547817602, -318.6955577907584143 ) ) ;
#32934=CARTESIAN_POINT ( 'NONE',  ( -8.712978146998754170, -284.6787398160598173, -339.9175775362199374 ) ) ;
#32935=DIRECTION ( 'NONE',  ( 0.000000000000000000, 0.000000000000000000, 1.000000000000000000 ) ) ;
#32936=CARTESIAN_POINT ( 'NONE',  ( -36.08578499355250102, -290.9567033222818964, -345.9235485338659259 ) ) ;
#32937=CARTESIAN_POINT ( 'NONE',  ( -108.4941548511755656, -294.2436177375766988, -294.2359434081013205 ) ) ;
#32938=CARTESIAN_POINT ( 'NONE',  ( 9.719935063024131239, -285.8786858023773902, -209.6210050987575926 ) ) ;
#32939=CARTESIAN_POINT ( 'NONE',  ( -103.1133941752558059, -289.4030812291434813, -236.7738166486678608 ) ) ;
#32941=CARTESIAN_POINT ( 'NONE',  ( 33.36778002442193269, -274.5006154486709988, -290.4424249614808673 ) ) ;
#32942=CARTESIAN_POINT ( 'NONE',  ( 18.89287927942060108, -292.3706590574209372, -318.8422044220893667 ) ) ;
#32944=DIRECTION ( 'NONE',  ( 0.000000000000000000, 0.000000000000000000, -1.000000000000000000 ) ) ;
#32945=CARTESIAN_POINT ( 'NONE',  ( -99.45531900679264936, -289.6244687465124912, -226.0372406331803745 ) ) ;
#32946=CARTESIAN_POINT ( 'NONE',  ( -62.85839590947979616, -287.3146177171687441, -201.0582291742840368 ) ) ;
#32947=CARTESIAN_POINT ( 'NONE',  ( 19.79593539477374620, -286.4789882025795009, -320.4732734816473680 ) ) ;
#32948=CARTESIAN_POINT ( 'NONE',  ( -84.03564565853366730, -286.8214501959630525, -213.4173926578460794 ) ) ;
#32950=CARTESIAN_POINT ( 'NONE',  ( -5.738135339045852490, -287.2814517793841560, -204.3638485644135301 ) ) ;
#32952=CARTESIAN_POINT ( 'NONE',  ( 35.11552575134603416, -295.2663892483308814, -249.6173644755602652 ) ) ;
#32953=CARTESIAN_POINT ( 'NONE',  ( -51.07533709564728497, -275.3062087946598240, -344.6625406541188568 ) ) ;
#32954=CARTESIAN_POINT ( 'NONE',  ( 33.00216862118396932, -276.2845747779161911, -301.6258652360431256 ) ) ;
#32955=CARTESIAN_POINT ( 'NONE',  ( -78.78380549637243746, -289.5787495064606105, -207.1173702057132573 ) ) ;
#32956=CARTESIAN_POINT ( 'NONE',  ( -112.0859179488524688, -278.7842186739925410, -251.8056194856152956 ) ) ;
#32957=CARTESIAN_POINT ( 'NONE',  ( -111.7363040177364724, -298.4454714529025523, -277.0720548665729552 ) ) ;
#32959=CARTESIAN_POINT ( 'NONE',  ( -110.6395504398199847, -271.5021483123970825, -270.3477634379551660 ) ) ;
#32960=CARTESIAN_POINT ( 'NONE',  ( -111.4024643768992746, -276.6166089877262948, -276.1520395222280513 ) ) ;
#32961=CARTESIAN_POINT ( 'NONE',  ( 19.56565204599082364, -278.8748759144665428, -221.4892127096036347 ) ) ;
#32963=CARTESIAN_POINT ( 'NONE',  ( 38.04765561763470316, -274.1850820714405472, -282.4885207786454657 ) ) ;
#32964=CARTESIAN_POINT ( 'NONE',  ( -108.2648688222162434, -297.8101774558010106, -290.3764095328523922 ) ) ;
#32965=CARTESIAN_POINT ( 'NONE',  ( 34.29385124588733191, -280.8205643207123217, -297.7443297823715511 ) ) ;
#32966=CARTESIAN_POINT ( 'NONE',  ( -63.64233483100957756, -296.3447099166472753, -338.7645706657486926 ) ) ;
#32967=CARTESIAN_POINT ( 'NONE',  ( -113.7402720745773905, -297.8048544962317123, -275.3241799979437019 ) ) ;
#32968=CARTESIAN_POINT ( 'NONE',  ( -78.86360831991031262, -273.1422962861992687, -210.2329151852054849 ) ) ;
#32969=CARTESIAN_POINT ( 'NONE',  ( -34.81472691223120108, -294.0840653066950949, -195.4036963493689711 ) ) ;
#32970=CARTESIAN_POINT ( 'NONE',  ( 20.28533836702271387, -287.0263233882139389, -219.2126126060300635 ) ) ;
#32971=CARTESIAN_POINT ( 'NONE',  ( 16.06741504395213482, -274.4445769333790395, -324.1723451437799213 ) ) ;
#32972=CARTESIAN_POINT ( 'NONE',  ( -3.062638987979901639, -288.4451890818139077, -339.3246112860156813 ) ) ;
#32974=CARTESIAN_POINT ( 'NONE',  ( 30.18335542718500619, -286.2301384233865065, -241.8788061238064984 ) ) ;
#32976=CARTESIAN_POINT ( 'NONE',  ( -111.8303938710173782, -288.4342144574989675, -279.5337173946844018 ) ) ;
#32978=CARTESIAN_POINT ( 'NONE',  ( -92.95696114837319612, -243.2523998898738569, -344.1903318997441374 ) ) ;
#32979=CARTESIAN_POINT ( 'NONE',  ( 28.28028695021345129, -287.4945350023901369, -302.4818784553601176 ) ) ;
#32981=CARTESIAN_POINT ( 'NONE',  ( -88.15678070623398810, -284.6840561578482038, -327.9703128154546334 ) ) ;
#32982=CARTESIAN_POINT ( 'NONE',  ( -11.22200553736694850, -291.4429814487121462, -198.1208881312806795 ) ) ;
#32983=CARTESIAN_POINT ( 'NONE',  ( -9.175955734774754902, -282.0144779793837984, -199.5576487280818299 ) ) ;
#32984=CARTESIAN_POINT ( 'NONE',  ( -39.58965874748531633, -281.3396790128235239, -193.8743323312287714 ) ) ;
#32985=CARTESIAN_POINT ( 'NONE',  ( -13.53137171193404065, -282.5676868547491267, -339.4224624954598539 ) ) ;
#32986=CARTESIAN_POINT ( 'NONE',  ( -48.89136816001263952, -279.1992999834397438, -344.5192820844910102 ) ) ;
#32987=CARTESIAN_POINT ( 'NONE',  ( -85.21641851755950370, -297.4114365667439870, -210.0534788385164973 ) ) ;
#32988=CARTESIAN_POINT ( 'NONE',  ( -11.33125291576214266, -275.7133156998286267, -201.5702580775294450 ) ) ;
#32989=CARTESIAN_POINT ( 'NONE',  ( -75.80603253352713011, -289.5564809184724027, -206.3293692086030262 ) ) ;
#32990=CARTESIAN_POINT ( 'NONE',  ( -52.68642951383230866, -296.7713645377598368, -198.6238324721507240 ) ) ;
#32992=DIRECTION ( 'NONE',  ( 0.000000000000000000, 0.000000000000000000, -1.000000000000000000 ) ) ;
#32993=CARTESIAN_POINT ( 'NONE',  ( -100.2348288785364048, -285.9314933304451642, -310.2792781458679201 ) ) ;
#32994=CARTESIAN_POINT ( 'NONE',  ( 29.31284564681175198, -295.1275702476369247, -308.3981541184227808 ) ) ;
#32995=CARTESIAN_POINT ( 'NONE',  ( -94.35931153799546678, -284.5577536097508755, -316.1290841247947014 ) ) ;
#32996=CARTESIAN_POINT ( 'NONE',  ( 16.78080552286736093, -275.3635927578397968, -324.8740543008594273 ) ) ;
#32997=CARTESIAN_POINT ( 'NONE',  ( -109.3812667624447528, -291.5459282934968996, -243.3092594025718256 ) ) ;
#32998=CARTESIAN_POINT ( 'NONE',  ( -96.59926540084762792, -283.3341574241499075, -223.1504577130137648 ) ) ;
#32999=CARTESIAN_POINT ( 'NONE',  ( -33.54465406605054767, -292.4320021119605144, -193.4759651065400021 ) ) ;
#33000=CARTESIAN_POINT ( 'NONE',  ( -110.1433600571587448, -290.8026839235597549, -276.6359475161144132 ) ) ;
#33003=CARTESIAN_POINT ( 'NONE',  ( 45.60988505783635105, 10.90853662155476123, -328.4231153613965830 ) ) ;
#33004=CARTESIAN_POINT ( 'NONE',  ( 19.28214613700657409, -283.7738104452764674, -321.5896715200768199 ) ) ;
#33005=CARTESIAN_POINT ( 'NONE',  ( 31.95455697924147032, -279.4809262143061233, -303.7686719486574702 ) ) ;
#33007=CARTESIAN_POINT ( 'NONE',  ( 26.73566498478314557, -279.9876221794355047, -234.7476745513384628 ) ) ;
#33008=CARTESIAN_POINT ( 'NONE',  ( -67.70417518725312789, -277.1065510281231354, -341.0991162568871573 ) ) ;
#33009=CARTESIAN_POINT ( 'NONE',  ( -96.24943387977992870, -281.1872334065592440, -224.1895642735208867 ) ) ;
#33010=CARTESIAN_POINT ( 'NONE',  ( -20.07155585692473210, -109.6737398891278872, -360.5847716769698650 ) ) ;
#33011=CARTESIAN_POINT ( 'NONE',  ( 27.79315718508426158, -280.6540538279702446, -310.4120297959395884 ) ) ;
#33012=CARTESIAN_POINT ( 'NONE',  ( -106.7525104449498770, -282.2114110230291431, -297.9607488108187567 ) ) ;
#33013=CARTESIAN_POINT ( 'NONE',  ( -112.6377882096997496, -274.5195184050028843, -261.9465711157578198 ) ) ;
#33014=CARTESIAN_POINT ( 'NONE',  ( -36.98895936933229223, -295.5399337075684798, -343.4342399511824624 ) ) ;
#33016=CARTESIAN_POINT ( 'NONE',  ( -19.93925799111839581, -290.9652209968617740, -198.9054221822963768 ) ) ;
#33017=CARTESIAN_POINT ( 'NONE',  ( -1.507864905510987619, -277.2411026900951470, -338.3997029187212888 ) ) ;
#33018=CARTESIAN_POINT ( 'NONE',  ( 23.05233286324211761, -274.9816108038741049, -229.3318581168621506 ) ) ;
#33019=CARTESIAN_POINT ( 'NONE',  ( 38.42438135388979248, -274.3223201608140585, -258.4023092643404311 ) ) ;
#33021=CARTESIAN_POINT ( 'NONE',  ( 33.42917534683050462, -273.2286666227298042, -245.3776858065712076 ) ) ;
#33024=CARTESIAN_POINT ( 'NONE',  ( 25.83236137166688096, -283.1417034202588638, -307.6537174318929146 ) ) ;
#33025=CARTESIAN_POINT ( 'NONE',  ( 21.74958287569445758, -283.9615763298186266, -318.1539726874498228 ) ) ;
#33026=CARTESIAN_POINT ( 'NONE',  ( -108.1252873150857567, -284.1415038273368054, -252.0970424947773267 ) ) ;
#33027=CARTESIAN_POINT ( 'NONE',  ( -1.094891457369224774, -274.9628548482588712, -334.7043125496806510 ) ) ;
#33028=CARTESIAN_POINT ( 'NONE',  ( -59.29111986838636028, -285.1995922600401627, -341.3312194994555853 ) ) ;
#33029=CARTESIAN_POINT ( 'NONE',  ( -79.04011402569013001, -276.1053380077994461, -331.1846851520571136 ) ) ;
#33031=CARTESIAN_POINT ( 'NONE',  ( -21.88219214424944781, -275.3346340096072140, -198.7006010605214499 ) ) ;
#33033=CARTESIAN_POINT ( 'NONE',  ( -113.6046712925309805, -279.2320628877154718, -280.1690514530494056 ) ) ;
#33037=CARTESIAN_POINT ( 'NONE',  ( -80.25835857444245391, -287.3385395835723557, -207.8600831769959427 ) ) ;
#33038=ADVANCED_FACE ( 'NONE', ( #81472 ), #76256, .T. ) ;
#33039=CARTESIAN_POINT ( 'NONE',  ( 3.898999922924293315, -293.6779872806772005, -330.7912957574439474 ) ) ;
#33040=CARTESIAN_POINT ( 'NONE',  ( -99.11774654396798212, -290.5105788848168231, -224.5456910706301983 ) ) ;
#33041=CARTESIAN_POINT ( 'NONE',  ( 27.26269421424738582, -285.3035601250166451, -234.1418532386952336 ) ) ;
#33042=CARTESIAN_POINT ( 'NONE',  ( -25.02548029837719668, -284.7868740185165279, -197.7581421543308977 ) ) ;
#33043=CARTESIAN_POINT ( 'NONE',  ( -104.4660478448649741, -289.2071674028874213, -239.1794574350610105 ) ) ;
#33044=CARTESIAN_POINT ( 'NONE',  ( -56.40733926150255684, -284.5084655308113497, -341.2387019435893762 ) ) ;
#33045=CARTESIAN_POINT ( 'NONE',  ( 36.26105334821276216, -273.3669764081778339, -255.9515609998747721 ) ) ;
#33046=CARTESIAN_POINT ( 'NONE',  ( -12.94040447992797382, -284.7639539793325412, -198.1737424588929457 ) ) ;
#33047=CARTESIAN_POINT ( 'NONE',  ( -59.58001654263917146, -299.7644559225720400, -198.6798162934733227 ) ) ;
#33048=CARTESIAN_POINT ( 'NONE',  ( 37.80770594883809110, -285.5313494615251102, -268.7501587031374584 ) ) ;
#33049=CARTESIAN_POINT ( 'NONE',  ( -46.49772091774341476, -280.8745014589430298, -197.6491612780373544 ) ) ;
#33050=CARTESIAN_POINT ( 'NONE',  ( -54.06826212402987153, -291.2664552886117804, -343.6965167060329804 ) ) ;
#33053=CARTESIAN_POINT ( 'NONE',  ( -83.28979008170658460, -297.5958328521694511, -330.4111278821402493 ) ) ;
#33055=CARTESIAN_POINT ( 'NONE',  ( -39.74036040608782372, -278.0218940935562273, -195.3866175647039256 ) ) ;
#33056=CARTESIAN_POINT ( 'NONE',  ( -13.90595589979413305, -291.5457240562551533, -197.1279067728692382 ) ) ;
#33057=CARTESIAN_POINT ( 'NONE',  ( -107.6374733117404361, -294.6553083425070554, -292.9976750377088592 ) ) ;
#33058=CARTESIAN_POINT ( 'NONE',  ( 35.18755864084348417, -280.3924270021191205, -282.2249327562059307 ) ) ;
#33059=CARTESIAN_POINT ( 'NONE',  ( -33.95109675677849737, -272.1749817370911728, -195.9983718758237501 ) ) ;
#33060=CARTESIAN_POINT ( 'NONE',  ( 34.12340519024993313, -294.6420029240479153, -253.1614981241125406 ) ) ;
#33061=CARTESIAN_POINT ( 'NONE',  ( -20.25526795762937127, -294.7662352645559167, -195.3538533559490702 ) ) ;
#33062=CARTESIAN_POINT ( 'NONE',  ( -104.6329770076042962, -295.5025213128503765, -234.2686448545316296 ) ) ;
#33064=CARTESIAN_POINT ( 'NONE',  ( -1.208053148290874734, -292.8194382752522529, -337.2214004581527433 ) ) ;
#33065=CARTESIAN_POINT ( 'NONE',  ( -103.3661617519135376, -291.5405758500167508, -302.8595084458196993 ) ) ;
#33067=CARTESIAN_POINT ( 'NONE',  ( -33.51018118450576821, -292.9044133253037785, -197.2875196018106294 ) ) ;
#33069=CARTESIAN_POINT ( 'NONE',  ( -3.651325501374625304, -280.6299759995120553, -337.7799476852829343 ) ) ;
#33070=CARTESIAN_POINT ( 'NONE',  ( 1.569833535611802722, -294.5164746057924390, -332.1858019889293132 ) ) ;
#33071=CARTESIAN_POINT ( 'NONE',  ( 0.8683584521353456820, -282.5570739756349781, -337.2268656555586404 ) ) ;
#33072=CARTESIAN_POINT ( 'NONE',  ( -35.90384704330953980, -282.7013356010795633, -347.3396578471469525 ) ) ;
#33073=CARTESIAN_POINT ( 'NONE',  ( 4.622124544456664985, -286.4845634646821964, -332.3837845326423235 ) ) ;
#33074=CARTESIAN_POINT ( 'NONE',  ( -114.4693872376281121, -273.8646567567205921, -270.3778293100139081 ) ) ;
#33075=CARTESIAN_POINT ( 'NONE',  ( -8.320669093651757109, -281.1590257665811237, -340.9897099980346411 ) ) ;
#33076=CARTESIAN_POINT ( 'NONE',  ( -17.81634514663873858, -287.7263923439008408, -344.5248087062251443 ) ) ;
#33078=CARTESIAN_POINT ( 'NONE',  ( 19.07512941299792075, -294.4836231006923413, -222.7840041404752753 ) ) ;
#33079=CARTESIAN_POINT ( 'NONE',  ( 32.48869680045604724, -277.3763901317145155, -301.3824325282109839 ) ) ;
#33080=CARTESIAN_POINT ( 'NONE',  ( -35.65805774584396914, -279.7405373823978607, -197.3469799397344957 ) ) ;
#33081=CARTESIAN_POINT ( 'NONE',  ( -42.05608268446400899, -292.1609478858293869, -193.5055742552185052 ) ) ;
#33082=CARTESIAN_POINT ( 'NONE',  ( -2.323627262914165215, -280.6722594902389005, -337.3166911144028859 ) ) ;
#33083=CARTESIAN_POINT ( 'NONE',  ( 32.97273632739031513, -292.8814269949173195, -290.8827005847365399 ) ) ;
#33084=CARTESIAN_POINT ( 'NONE',  ( -110.6556608729419509, -294.3489524138628894, -286.1745240955714280 ) ) ;
#33087=CARTESIAN_POINT ( 'NONE',  ( 6.094495920175158510, -293.9526385777739961, -329.1718042848390269 ) ) ;
#33089=CARTESIAN_POINT ( 'NONE',  ( -92.05005921254146983, -282.6952119285918457, -226.6919474004047572 ) ) ;
#33090=CARTESIAN_POINT ( 'NONE',  ( -14.88359410320592957, -297.3856292487311066, -193.5998961811205561 ) ) ;
#33091=CARTESIAN_POINT ( 'NONE',  ( 20.14462282524261028, -279.0145978632019137, -220.9892991889750533 ) ) ;
#33092=CARTESIAN_POINT ( 'NONE',  ( -73.39552163992144074, -286.8996886490954807, -202.8234010165467680 ) ) ;
#33093=CARTESIAN_POINT ( 'NONE',  ( -48.06307987884917310, -289.0255318033749177, -342.6205331511768009 ) ) ;
#33094=CARTESIAN_POINT ( 'NONE',  ( -48.69574212002144264, -278.7193387639670163, -343.2264087052357695 ) ) ;
#33095=CARTESIAN_POINT ( 'NONE',  ( -70.47636386213999060, -293.5113093754877127, -337.2486419758903367 ) ) ;
#33096=CARTESIAN_POINT ( 'NONE',  ( -105.1224510126624949, -274.5418370036176157, -241.0388890186827950 ) ) ;
#33098=CARTESIAN_POINT ( 'NONE',  ( -71.85439456126579216, -276.3139440544882177, -335.1518687466526103 ) ) ;
#33100=CARTESIAN_POINT ( 'NONE',  ( 76.35222964319555672, -299.1058724536635509, -193.3884058114072388 ) ) ;
#33101=CARTESIAN_POINT ( 'NONE',  ( -69.35554290129813637, -291.3968966467350583, -337.5654933820780457 ) ) ;
#33102=CARTESIAN_POINT ( 'NONE',  ( 8.441914161598603528, -296.0370118720466053, -331.2733587559479247 ) ) ;
#33105=CARTESIAN_POINT ( 'NONE',  ( -100.3876663733047252, -290.6950065729685662, -307.4621349646194517 ) ) ;
#33108=CARTESIAN_POINT ( 'NONE',  ( -113.2901850105230466, -297.3554776023441377, -258.2302207225033612 ) ) ;
#33109=CARTESIAN_POINT ( 'NONE',  ( -101.2719468598982928, -288.1490014129813630, -311.1176275136417644 ) ) ;
#33111=CARTESIAN_POINT ( 'NONE',  ( -68.17288964948761532, -297.9916296626012127, -199.7693638474820830 ) ) ;
#33114=CARTESIAN_POINT ( 'NONE',  ( -106.6389794118234562, -292.4860736968058745, -238.2884066506962597 ) ) ;
#33115=CARTESIAN_POINT ( 'NONE',  ( -115.3430155898818299, -287.2662352645559167, -252.5904736702033517 ) ) ;
#33116=CARTESIAN_POINT ( 'NONE',  ( -106.9090814665903793, -286.1908228946193731, -298.0775466192001772 ) ) ;
#33117=CARTESIAN_POINT ( 'NONE',  ( 0.3998229562577181873, -272.5559825928079931, -205.7272299721121556 ) ) ;
#33118=CARTESIAN_POINT ( 'NONE',  ( -100.5152130761826186, -275.0052284895160710, -230.9857264471263250 ) ) ;
#33119=CARTESIAN_POINT ( 'NONE',  ( -97.91922718657802704, -289.2258106236884032, -227.0110789502120667 ) ) ;
#33120=CARTESIAN_POINT ( 'NONE',  ( -41.29590191099759267, -278.9618188557272447, -346.0356625295015647 ) ) ;
#33122=CARTESIAN_POINT ( 'NONE',  ( 17.06281253990017532, -280.8557823844755603, -221.6872132557001294 ) ) ;
#33123=CARTESIAN_POINT ( 'NONE',  ( 18.04718183035087264, -280.2220641233119522, -222.6348310530956383 ) ) ;
#33124=CARTESIAN_POINT ( 'NONE',  ( 10.34464992864179500, -277.4915762735131466, -330.4914449567640418 ) ) ;
#33125=CARTESIAN_POINT ( 'NONE',  ( -35.33099143948599163, -278.8717622486105370, -193.7715137033361827 ) ) ;
#33126=CARTESIAN_POINT ( 'NONE',  ( -78.45397945840984733, -207.3402917149092843, -354.1116341293970891 ) ) ;
#33127=CARTESIAN_POINT ( 'NONE',  ( 37.36566509161409755, -276.7155043873352156, -288.0708150203219589 ) ) ;
#33129=CARTESIAN_POINT ( 'NONE',  ( -36.96279093540193372, -275.5769624299149996, -194.0424553924729310 ) ) ;
#33130=CARTESIAN_POINT ( 'NONE',  ( -53.35057174420112602, -276.3376638359844719, -200.3683826091709648 ) ) ;
#33133=CARTESIAN_POINT ( 'NONE',  ( 18.89005616163744605, -287.9668141813629632, -223.3073691477756597 ) ) ;
#33134=CARTESIAN_POINT ( 'NONE',  ( 2.194386335091289109, -288.3341391797164306, -205.4698868318808991 ) ) ;
#33135=CARTESIAN_POINT ( 'NONE',  ( -106.6653291487429556, -290.2084013814618402, -247.1635507058722112 ) ) ;
#33136=CARTESIAN_POINT ( 'NONE',  ( -30.88276599135153688, -285.6393417142027147, -193.6809630047584676 ) ) ;
#33138=CARTESIAN_POINT ( 'NONE',  ( 26.23800227585467582, -280.4623352022327367, -307.9328669103387028 ) ) ;
#33139=CARTESIAN_POINT ( 'NONE',  ( 31.64163917898076051, -289.7750386339739066, -297.9254880904029505 ) ) ;
#33140=CARTESIAN_POINT ( 'NONE',  ( -48.45213739287968480, -281.6760186174969363, -343.2121024294415292 ) ) ;
#33141=CARTESIAN_POINT ( 'NONE',  ( -89.83748714940942648, -280.6074712480287872, -218.8551773005068242 ) ) ;
#33142=CARTESIAN_POINT ( 'NONE',  ( 15.64682387207299818, -276.7689712314507346, -320.6622587843362453 ) ) ;
#33143=CARTESIAN_POINT ( 'NONE',  ( -112.1807189268762954, -289.1416171884576443, -286.7052296321610356 ) ) ;
#33144=CARTESIAN_POINT ( 'NONE',  ( -73.54598975211922607, -286.3874300006120848, -202.5274969870066570 ) ) ;
#33145=CARTESIAN_POINT ( 'NONE',  ( -4.805674683699147742, -286.9616232467326427, -200.6407195914692352 ) ) ;
#33146=CARTESIAN_POINT ( 'NONE',  ( 9.910312051490468122, -282.5468458581152049, -326.0715290498166610 ) ) ;
#33149=CARTESIAN_POINT ( 'NONE',  ( -112.4450284264164281, -292.5444324235590443, -259.9863624170432104 ) ) ;
#33150=CARTESIAN_POINT ( 'NONE',  ( -70.66767281404656842, -290.3066292962160446, -201.4940153883243852 ) ) ;
#33151=CARTESIAN_POINT ( 'NONE',  ( 3.069734774904482322, -273.6679745993777715, -209.2241232902831314 ) ) ;
#33152=CARTESIAN_POINT ( 'NONE',  ( -111.1199406074225919, -295.6278934692866756, -292.0890015627458070 ) ) ;
#33153=CARTESIAN_POINT ( 'NONE',  ( -38.89294845073587226, -290.5122174202311953, -196.6841108303447925 ) ) ;
#33154=CARTESIAN_POINT ( 'NONE',  ( -58.72208927509728937, -293.5723461906366083, -341.2190954549542425 ) ) ;
#33155=CARTESIAN_POINT ( 'NONE',  ( -78.38380932092603359, -290.8228228185203648, -331.2719119771732039 ) ) ;
#33157=CARTESIAN_POINT ( 'NONE',  ( -110.9012812813950575, -292.3636499936778819, -285.0544567425449145 ) ) ;
#33158=CARTESIAN_POINT ( 'NONE',  ( -7.884618368823592682, -290.4370185387188599, -201.1928959562539205 ) ) ;
#33159=CARTESIAN_POINT ( 'NONE',  ( -80.89647905448541110, -297.6431033639914290, -331.4813995521877814 ) ) ;
#33160=CARTESIAN_POINT ( 'NONE',  ( -5.707835343663168359, -287.4198487686622343, -204.2964989815021681 ) ) ;
#33161=CARTESIAN_POINT ( 'NONE',  ( -30.02423387210372852, -276.1242252469000391, -195.3620413895717718 ) ) ;
#33162=CARTESIAN_POINT ( 'NONE',  ( -9.371169638907522526, -275.4894771109472913, -341.6749184898459362 ) ) ;
#33163=CARTESIAN_POINT ( 'NONE',  ( -97.21408223664178649, -296.3961389958371342, -222.2003800102980904 ) ) ;
#33164=CARTESIAN_POINT ( 'NONE',  ( -29.62982346885026530, -275.1931643009767754, -344.0231973670973389 ) ) ;
#33165=CARTESIAN_POINT ( 'NONE',  ( -69.11619310425287210, -277.7107528691086600, -203.0432466714617021 ) ) ;
#33166=CARTESIAN_POINT ( 'NONE',  ( -68.46484161296314142, -274.8389907444129676, -203.8756922473113775 ) ) ;
#33167=CARTESIAN_POINT ( 'NONE',  ( -12.15009062969877895, -275.1297510472127783, -342.3318467207231492 ) ) ;
#33169=CARTESIAN_POINT ( 'NONE',  ( -109.2314900355806628, -273.3817762121369697, -256.8330798644309994 ) ) ;
#33172=CARTESIAN_POINT ( 'NONE',  ( -18.16769952643022634, -286.8263164446934184, -343.2361102695281261 ) ) ;
#33173=CARTESIAN_POINT ( 'NONE',  ( 30.17562777812529617, -275.0118763886091529, -242.4721066380130026 ) ) ;
#33174=CARTESIAN_POINT ( 'NONE',  ( 20.57290064324190126, -288.2388450483110205, -321.1244443137596249 ) ) ;
#33176=CARTESIAN_POINT ( 'NONE',  ( -31.83253012887607980, -288.6512782657153480, -347.1951243307299819 ) ) ;
#33177=CARTESIAN_POINT ( 'NONE',  ( -32.07894891472518140, -300.0976079745157108, -195.0041440767023744 ) ) ;
#33178=CARTESIAN_POINT ( 'NONE',  ( 21.96085315542601890, -292.1788802332337127, -316.0245657363597616 ) ) ;
#33179=CARTESIAN_POINT ( 'NONE',  ( 21.85286100594614567, -280.0893759962342529, -221.3696620610721766 ) ) ;
#33181=CARTESIAN_POINT ( 'NONE',  ( -59.32065368257949700, -277.7676009466405844, -198.6004912461297067 ) ) ;
#33183=CARTESIAN_POINT ( 'NONE',  ( -61.39957090083058944, -288.1666413433127332, -339.7033804084038593 ) ) ;
#33186=CARTESIAN_POINT ( 'NONE',  ( -92.20530673716717729, -289.2679089803717147, -219.2052097926309955 ) ) ;
#33187=CARTESIAN_POINT ( 'NONE',  ( -63.57142563311793282, -275.2241214385912258, -201.4801639173576007 ) ) ;
#33188=CARTESIAN_POINT ( 'NONE',  ( 6.601100826818031564, -283.8932888353776320, -332.9369214624183542 ) ) ;
#33189=CARTESIAN_POINT ( 'NONE',  ( -35.84299033034217530, -296.0909377233871282, -195.0064122322097262 ) ) ;
#33190=CARTESIAN_POINT ( 'NONE',  ( -109.9944159237722658, -284.6525547848441988, -262.7500509422749815 ) ) ;
#33191=CARTESIAN_POINT ( 'NONE',  ( 20.30584824956651957, -276.3367230657516984, -224.6010986315913840 ) ) ;
#33192=CARTESIAN_POINT ( 'NONE',  ( 26.77312003911535854, -275.8734086592781409, -235.0150759722817213 ) ) ;
#33193=CARTESIAN_POINT ( 'NONE',  ( -1.313224155831289597, -284.5744958153852053, -336.1552240957446429 ) ) ;
#33194=CARTESIAN_POINT ( 'NONE',  ( -35.79735738312007243, -297.1306974705111088, -197.1260763546636383 ) ) ;
#33197=CARTESIAN_POINT ( 'NONE',  ( 39.50199093484781798, -293.4565105467999047, -276.0412605930700920 ) ) ;
#33198=CARTESIAN_POINT ( 'NONE',  ( -74.39349363484268451, -287.5368150357599006, -205.5465134418000730 ) ) ;
#33200=CARTESIAN_POINT ( 'NONE',  ( 31.09738932201053885, -296.4086741954486115, -195.3901485728259502 ) ) ;
#33201=CARTESIAN_POINT ( 'NONE',  ( -111.6738409199724629, -277.5045736829874272, -289.8779844555725731 ) ) ;
#33202=CARTESIAN_POINT ( 'NONE',  ( -98.40045421182952623, -288.3389419493095147, -315.9707378627116441 ) ) ;
#33203=CARTESIAN_POINT ( 'NONE',  ( -61.74624149085314428, -284.8951274314487705, -339.9499248228096349 ) ) ;
#33204=CARTESIAN_POINT ( 'NONE',  ( -18.74092857068766094, -278.5694756802828351, -341.9989941966868514 ) ) ;
#33205=CARTESIAN_POINT ( 'NONE',  ( -1.263912643127763191, -287.9464861505516637, -203.0038648904761089 ) ) ;
#33206=CARTESIAN_POINT ( 'NONE',  ( -65.59245829820396523, -281.6828876231624577, -200.8852566155559884 ) ) ;
#33207=CARTESIAN_POINT ( 'NONE',  ( -32.68472395937533292, -274.2759688540571688, -193.4889237914557896 ) ) ;
#33208=CARTESIAN_POINT ( 'NONE',  ( -112.4848703791476083, -278.1752677026754554, -287.1689723713978424 ) ) ;
#33209=CARTESIAN_POINT ( 'NONE',  ( -31.46474598745840723, -296.8976669832055109, -344.6198714485938126 ) ) ;
#33210=DIRECTION ( 'NONE',  ( 0.000000000000000000, 0.000000000000000000, 1.000000000000000000 ) ) ;
#33212=CARTESIAN_POINT ( 'NONE',  ( -104.7001572184116753, -271.2530539699363885, -235.0791172798350033 ) ) ;
#33213=CARTESIAN_POINT ( 'NONE',  ( 27.91906468313075607, -274.6143612140683672, -237.5126626503203227 ) ) ;
#33214=CARTESIAN_POINT ( 'NONE',  ( -35.84949538551849457, -299.1500887552125505, -193.6699611145742210 ) ) ;
#33215=CARTESIAN_POINT ( 'NONE',  ( 35.96713779180102222, -289.4460535570865432, -280.6412464792344394 ) ) ;
#33216=CARTESIAN_POINT ( 'NONE',  ( -113.5402016165382548, -298.0097694524600342, -275.3138384975532063 ) ) ;
#33217=CARTESIAN_POINT ( 'NONE',  ( -109.9643658699752393, -297.4487345068091031, -294.7323538720502825 ) ) ;
#33218=CARTESIAN_POINT ( 'NONE',  ( -111.5208389929369162, -292.6843288237747061, -260.1024113009410144 ) ) ;
#33219=CARTESIAN_POINT ( 'NONE',  ( -99.50262570966383180, -277.1176352740963580, -228.6032428094024453 ) ) ;
#33220=CARTESIAN_POINT ( 'NONE',  ( -110.4530485355167997, -280.2903059248055229, -284.4299598767115640 ) ) ;
#33221=CARTESIAN_POINT ( 'NONE',  ( -84.97793486829843346, -295.4692572898205754, -213.0915344157571951 ) ) ;
#33222=CARTESIAN_POINT ( 'NONE',  ( -93.46793609787764012, -285.7096954792746715, -321.2738799542651122 ) ) ;
#33223=CARTESIAN_POINT ( 'NONE',  ( 2.627008637653146295, -285.5224890690780057, -208.9060254940336847 ) ) ;
#33224=CARTESIAN_POINT ( 'NONE',  ( -111.9030559682143604, -274.5283560713371003, -270.3862797920663752 ) ) ;
#33226=CARTESIAN_POINT ( 'NONE',  ( 34.54175682619548837, -287.3881966606786023, -283.2007481613696882 ) ) ;
#33228=CARTESIAN_POINT ( 'NONE',  ( 6.758540737419452604, -283.5477435763236826, -333.1688832126113766 ) ) ;
#33229=CARTESIAN_POINT ( 'NONE',  ( -110.3628441122352086, -272.8853797144980717, -270.3653515045655240 ) ) ;
#33230=CARTESIAN_POINT ( 'NONE',  ( -40.78319162524128672, -284.8048307975259945, -193.7836104478722064 ) ) ;
#33231=CARTESIAN_POINT ( 'NONE',  ( -31.10486643115158145, -281.0702406907684576, -193.7976601323755403 ) ) ;
#33232=CARTESIAN_POINT ( 'NONE',  ( -72.20744052326691076, -281.1195901126344552, -202.4710646483769665 ) ) ;
#33233=CARTESIAN_POINT ( 'NONE',  ( 27.83118925510074249, -281.3477514490717226, -229.2949179761089624 ) ) ;
#33235=CARTESIAN_POINT ( 'NONE',  ( 27.36219212280433055, -290.6237833571632905, -239.2376011013261916 ) ) ;
#33236=CARTESIAN_POINT ( 'NONE',  ( -55.75868456242086779, -169.6758193678651025, -364.5828727736617338 ) ) ;
#33238=CARTESIAN_POINT ( 'NONE',  ( -84.36181329012404717, -275.4034827085500865, -212.1448197354905005 ) ) ;
#33239=CARTESIAN_POINT ( 'NONE',  ( 138.2325648905753610, 180.7664419875970623, -241.1855197640491042 ) ) ;
#33241=CARTESIAN_POINT ( 'NONE',  ( 35.36815920766267851, -279.3544182253640429, -253.4755276013975163 ) ) ;
#33242=CARTESIAN_POINT ( 'NONE',  ( 36.12269179020163534, -295.5585899757391530, -289.7765019833174733 ) ) ;
#33243=CARTESIAN_POINT ( 'NONE',  ( -82.42919066686779672, -295.0348199151614494, -327.9670460734145649 ) ) ;
#33244=CARTESIAN_POINT ( 'NONE',  ( -81.88964679804441005, -290.9705478309996920, -207.6314810430274918 ) ) ;
#33245=CARTESIAN_POINT ( 'NONE',  ( -82.08642841123406697, -219.1949203529281647, -349.1242040296514233 ) ) ;
#33246=CARTESIAN_POINT ( 'NONE',  ( -113.0711862319940906, -294.9936823940829527, -280.9302372399137653 ) ) ;
#33247=CARTESIAN_POINT ( 'NONE',  ( 30.70725159432555884, -285.5713680761861610, -241.6668162570057063 ) ) ;
#33248=CARTESIAN_POINT ( 'NONE',  ( 17.63729207669877752, -294.7089755207845201, -220.4041347016804195 ) ) ;
#33249=CARTESIAN_POINT ( 'NONE',  ( -109.1987232286076193, -285.6644807543817706, -285.8419717287972048 ) ) ;
#33251=CARTESIAN_POINT ( 'NONE',  ( 38.37619317294442567, -294.6528920351498186, -283.0749528449060790 ) ) ;
#33252=CARTESIAN_POINT ( 'NONE',  ( 34.00186220612027199, -282.2521035225376522, -286.1118181365835653 ) ) ;
#33253=CARTESIAN_POINT ( 'NONE',  ( -112.9949607925361477, -295.4992883555790968, -258.2534469423519567 ) ) ;
#33254=CARTESIAN_POINT ( 'NONE',  ( -95.32970853143022794, -290.6720971471866051, -320.7749028260804494 ) ) ;
#33255=CARTESIAN_POINT ( 'NONE',  ( -96.53554474093061799, -291.7060953118628959, -221.1918430935569688 ) ) ;
#33256=CARTESIAN_POINT ( 'NONE',  ( -0.9896000240085451871, -288.7222066576974271, -333.7243181166660406 ) ) ;
#33259=CARTESIAN_POINT ( 'NONE',  ( -83.41498438703072793, -297.5361043359898758, -330.5733874343066532 ) ) ;
#33260=CARTESIAN_POINT ( 'NONE',  ( 18.95429746841130481, -297.4279038174026937, -193.8665315653600203 ) ) ;
#33261=CARTESIAN_POINT ( 'NONE',  ( -36.99522110494318383, -279.1153423193426306, -197.1266424861778717 ) ) ;
#33263=CARTESIAN_POINT ( 'NONE',  ( 15.98889792291381973, -274.2917707236242109, -214.9050613733796240 ) ) ;
#33264=CARTESIAN_POINT ( 'NONE',  ( -71.97387426953163470, -296.0654448987113483, -205.2981877105294757 ) ) ;
#33265=CARTESIAN_POINT ( 'NONE',  ( -13.36439972901751183, -278.5980054456549624, -340.6715107450201572 ) ) ;
#33266=CARTESIAN_POINT ( 'NONE',  ( -35.33356310345696016, -272.2171734265552345, -196.1403635641506469 ) ) ;
#33267=CARTESIAN_POINT ( 'NONE',  ( 1.794469701624061608, -295.7213561357832532, -332.5139165581019824 ) ) ;
#33268=CARTESIAN_POINT ( 'NONE',  ( -90.27855973992070915, -298.3612535637203678, -219.5744042969455450 ) ) ;
#33269=DIRECTION ( 'NONE',  ( 1.000000000000000000, 0.000000000000000000, 0.000000000000000000 ) ) ;
#33270=CARTESIAN_POINT ( 'NONE',  ( -105.2355543238093105, -297.7007546666828262, -305.0730266092111265 ) ) ;
#33271=CARTESIAN_POINT ( 'NONE',  ( -34.11881225684701491, -296.0922507526707932, -195.1955383508204989 ) ) ;
#33272=CARTESIAN_POINT ( 'NONE',  ( -55.04505863320998316, -292.4698269058708888, -199.4352146363740133 ) ) ;
#33273=CARTESIAN_POINT ( 'NONE',  ( -108.3154105057184324, -289.3817303103195968, -250.9161352504875708 ) ) ;
#33275=CARTESIAN_POINT ( 'NONE',  ( -24.17631111011271372, -274.7081597337451626, -194.5033055658255137 ) ) ;
#33277=CARTESIAN_POINT ( 'NONE',  ( -92.91516337080851429, -273.3922917929315304, -223.0069486626450157 ) ) ;
#33279=CARTESIAN_POINT ( 'NONE',  ( 7.546099883699421085, -282.6406099732241159, -209.7694807524165412 ) ) ;
#33280=CARTESIAN_POINT ( 'NONE',  ( 0.6090892985368842050, -281.2421122378731297, -336.8069355093072090 ) ) ;
#33281=CARTESIAN_POINT ( 'NONE',  ( -71.53299156402339065, -276.8405610880930112, -339.2397676284468844 ) ) ;
#33282=CARTESIAN_POINT ( 'NONE',  ( -108.5848795113629279, -283.5295897961786409, -287.0595393189416882 ) ) ;
#33283=CARTESIAN_POINT ( 'NONE',  ( 10.31021374610265617, -280.3967150952920520, -328.5604030506088407 ) ) ;
#33284=CARTESIAN_POINT ( 'NONE',  ( -51.65846654883972633, -272.4402773672729268, -198.1257770416210064 ) ) ;
#33285=CARTESIAN_POINT ( 'NONE',  ( -100.5170368329778654, -280.0069898695990673, -310.8772668099807674 ) ) ;
#33288=CARTESIAN_POINT ( 'NONE',  ( -37.23224573514328029, -296.2933724657740981, -194.3737234103267610 ) ) ;
#33289=CARTESIAN_POINT ( 'NONE',  ( -66.96213998607029794, -279.4396156112838412, -339.4455443851739460 ) ) ;
#33291=CARTESIAN_POINT ( 'NONE',  ( -94.73903062906690309, -287.1486480005538056, -221.1413844251751186 ) ) ;
#33293=CARTESIAN_POINT ( 'NONE',  ( 12.07965199447950333, -284.7387967406844496, -213.8789230781245294 ) ) ;
#33295=CARTESIAN_POINT ( 'NONE',  ( -95.93051517134986739, -294.7291850124621533, -314.5913427779823337 ) ) ;
#33296=CARTESIAN_POINT ( 'NONE',  ( -99.89513648522047617, -288.1480376965180312, -310.3352731273910194 ) ) ;
#33298=CARTESIAN_POINT ( 'NONE',  ( -93.71022004583248588, -293.8646530673283905, -319.8342481949042053 ) ) ;
#33299=CARTESIAN_POINT ( 'NONE',  ( -1.279973881134012892, -285.0015678461560924, -203.1133696635105821 ) ) ;
#33300=CARTESIAN_POINT ( 'NONE',  ( 32.11436023637819659, -283.4826781829265201, -295.4581956494556039 ) ) ;
#33301=CARTESIAN_POINT ( 'NONE',  ( 36.01273878315765131, -279.5398482319560003, -250.4849618751943012 ) ) ;
#33302=CARTESIAN_POINT ( 'NONE',  ( -39.95803529557185385, -289.0858085025106448, -343.3637959310983092 ) ) ;
#33303=CARTESIAN_POINT ( 'NONE',  ( -6.539217865572089394, -281.8900256738776307, -203.5148712634754418 ) ) ;
#33304=CARTESIAN_POINT ( 'NONE',  ( -14.26762284225651101, -281.1618676301493451, -200.8799844823172975 ) ) ;
#33305=CARTESIAN_POINT ( 'NONE',  ( 26.07453879285593956, -290.0787510398249651, -311.1610326075498847 ) ) ;
#33308=CARTESIAN_POINT ( 'NONE',  ( -97.81306561133810362, -273.1897003597648563, -222.6933725293671387 ) ) ;
#33310=CARTESIAN_POINT ( 'NONE',  ( -98.11486664206425701, -293.1252269755775046, -226.9323422131175789 ) ) ;
#33312=CARTESIAN_POINT ( 'NONE',  ( 40.64545035920995986, -289.8376638359844719, -252.5284128619064461 ) ) ;
#33314=CARTESIAN_POINT ( 'NONE',  ( -15.15571491175780139, -274.7654898972930368, -342.2335063922344602 ) ) ;
#33316=CARTESIAN_POINT ( 'NONE',  ( -33.49580821277195497, -293.4044070935761965, -346.4769890068221798 ) ) ;
#33317=CARTESIAN_POINT ( 'NONE',  ( -96.92929790717360561, -296.6496484692112858, -228.0845685411242414 ) ) ;
#33318=CARTESIAN_POINT ( 'NONE',  ( -78.54620054423907050, -291.1378183172272998, -331.5199785405384318 ) ) ;
#33319=CARTESIAN_POINT ( 'NONE',  ( -66.94456868883817435, -285.2056502369458713, -338.2102950118643889 ) ) ;
#33320=CARTESIAN_POINT ( 'NONE',  ( -40.62540460323569391, -293.4369119084665840, -194.0078535165154392 ) ) ;
#33321=CARTESIAN_POINT ( 'NONE',  ( -53.30289070689140374, -293.1668951046262350, -195.4835838815039040 ) ) ;
#33322=CARTESIAN_POINT ( 'NONE',  ( -44.23282153925701010, -287.9651449196662725, -195.6783683398700475 ) ) ;
#33323=CARTESIAN_POINT ( 'NONE',  ( -33.91739589480346240, -280.2607953581726861, -193.4372975818709790 ) ) ;
#33324=CARTESIAN_POINT ( 'NONE',  ( -91.67877995074051967, -293.8990658326607672, -322.8663172855614221 ) ) ;
#33325=CARTESIAN_POINT ( 'NONE',  ( -2.894744918062149619, -282.4428947460176573, -339.2409094122591000 ) ) ;
#33326=CARTESIAN_POINT ( 'NONE',  ( 35.58252660151414659, -277.2323909383133582, -256.4714585798574262 ) ) ;
#33327=CARTESIAN_POINT ( 'NONE',  ( -37.30987171927208124, -297.5519495502701943, -345.3611179825600175 ) ) ;
#33328=CARTESIAN_POINT ( 'NONE',  ( -42.74215459161417385, -275.2592040953476271, -345.9332065636634752 ) ) ;
#33330=CARTESIAN_POINT ( 'NONE',  ( 19.72801145091433028, -280.4158735269139129, -224.7427394254780211 ) ) ;
#33331=CARTESIAN_POINT ( 'NONE',  ( -109.3581844763485691, -279.4239997028773246, -296.6243382251321350 ) ) ;
#33332=CARTESIAN_POINT ( 'NONE',  ( -80.79511299287010218, -284.5373227655552455, -207.0148866303880482 ) ) ;
#33333=CARTESIAN_POINT ( 'NONE',  ( 21.79006443254570158, -294.6957335035034475, -225.8481037547746837 ) ) ;
#33334=CARTESIAN_POINT ( 'NONE',  ( 37.15888309450676275, -276.9492518119720330, -254.2962741974701828 ) ) ;
#33335=CARTESIAN_POINT ( 'NONE',  ( 32.57592333003917417, -277.2663095709509093, -301.4227374096849417 ) ) ;
#33336=CYLINDRICAL_SURFACE ( 'NONE', #65635, 6.654241149514406040 ) ;
#33337=CARTESIAN_POINT ( 'NONE',  ( 35.10581063041140482, -275.5090417618965262, -279.7284396159415110 ) ) ;
#33338=CARTESIAN_POINT ( 'NONE',  ( -56.24235770193362072, -297.2962361136173399, -342.8219490355584753 ) ) ;
#33339=CARTESIAN_POINT ( 'NONE',  ( -92.86478474100206881, -283.2536745913792515, -220.1131485881716401 ) ) ;
#33340=CARTESIAN_POINT ( 'NONE',  ( 21.29709704572013607, -292.5461031493408655, -220.4687846005323024 ) ) ;
#33341=CARTESIAN_POINT ( 'NONE',  ( 38.17965917425229350, -289.0240411683405455, -260.2139654669492757 ) ) ;
#33342=CARTESIAN_POINT ( 'NONE',  ( 34.52222263106197175, -292.2822080820232031, -255.8765510184112770 ) ) ;
#33344=CARTESIAN_POINT ( 'NONE',  ( -53.24879693982099838, -290.4268897770492686, -195.5703648430829276 ) ) ;
#33345=CARTESIAN_POINT ( 'NONE',  ( -36.20154351210599231, -291.7335187045921430, -197.3363956435701709 ) ) ;
#33347=CARTESIAN_POINT ( 'NONE',  ( -71.75538951252248410, -290.5759539253356252, -338.8971704947978765 ) ) ;
#33348=CARTESIAN_POINT ( 'NONE',  ( -108.5059141385938375, -278.6689131510411812, -286.7793455013163566 ) ) ;
#33349=CARTESIAN_POINT ( 'NONE',  ( -101.3777752111107446, -294.9142812390116433, -312.6575827542811794 ) ) ;
#33350=CARTESIAN_POINT ( 'NONE',  ( -103.9563095375059163, -285.7048217864644357, -231.8389788811792585 ) ) ;
#33351=CARTESIAN_POINT ( 'NONE',  ( -32.31204088466856206, -286.4471958295074501, -193.5335893367187339 ) ) ;
#33352=CARTESIAN_POINT ( 'NONE',  ( -34.84156663645412522, -283.3532007187520776, -343.3518892696752118 ) ) ;
#33353=CARTESIAN_POINT ( 'NONE',  ( 167.7576066075372410, 232.6804878302470740, -192.6587424375081241 ) ) ;
#33354=CARTESIAN_POINT ( 'NONE',  ( -23.37133263859758614, -107.7079578404835019, -361.6456582812304532 ) ) ;
#33355=CARTESIAN_POINT ( 'NONE',  ( 172.3370473676889389, 241.3813337058840318, -177.2540278754750886 ) ) ;
#33356=CARTESIAN_POINT ( 'NONE',  ( 28.17055419427044782, -275.1913368517148797, -303.0443929753960788 ) ) ;
#33357=CARTESIAN_POINT ( 'NONE',  ( -24.28801029419035729, -275.8020263774093905, -342.5503431574682622 ) ) ;
#33358=CARTESIAN_POINT ( 'NONE',  ( -103.7934878644902739, -296.5659724116084135, -231.4787383676991226 ) ) ;
#33359=CARTESIAN_POINT ( 'NONE',  ( -37.84230186231246762, -140.7305523473693540, -361.6245629116337454 ) ) ;
#33360=CARTESIAN_POINT ( 'NONE',  ( 24.09393627825123829, -273.6268531445568897, -224.7654948012895204 ) ) ;
#33361=CARTESIAN_POINT ( 'NONE',  ( -24.44154745801118267, -275.9790657714007693, -197.4283655155201700 ) ) ;
#33362=CARTESIAN_POINT ( 'NONE',  ( -36.20080988378119002, -299.0073551978468913, -193.5962329938457174 ) ) ;
#33363=CARTESIAN_POINT ( 'NONE',  ( 33.76875860297097631, -287.8227272751017267, -253.5353332559716648 ) ) ;
#33364=CARTESIAN_POINT ( 'NONE',  ( -113.0429952711294419, -297.1861496475119111, -283.8324629488006394 ) ) ;
#33365=CARTESIAN_POINT ( 'NONE',  ( -107.7192806993222405, -297.4429453158240904, -239.1404177300734659 ) ) ;
#33366=CARTESIAN_POINT ( 'NONE',  ( -20.84611114343226390, -295.0012953506719100, -341.5250754459366931 ) ) ;
#33368=CARTESIAN_POINT ( 'NONE',  ( 6.381432469543416808, -276.5606396297720835, -208.6722360647949586 ) ) ;
#33372=CARTESIAN_POINT ( 'NONE',  ( -7.555020132883479178, -279.9399520094541458, -199.4082565219720777 ) ) ;
#33373=CARTESIAN_POINT ( 'NONE',  ( -13.69813227323517779, -277.6789896027577242, -339.7281388262501309 ) ) ;
#33374=CARTESIAN_POINT ( 'NONE',  ( 33.25128739806281430, -277.6753685026446306, -298.6207676605339998 ) ) ;
#33375=CARTESIAN_POINT ( 'NONE',  ( -100.7274125782280549, -276.0248484130926840, -311.2075551554477784 ) ) ;
#33376=CARTESIAN_POINT ( 'NONE',  ( -103.2632956835919629, -273.4701660895620421, -238.8598214874925532 ) ) ;
#33377=CARTESIAN_POINT ( 'NONE',  ( -109.7249761294971364, -294.9523377310999308, -283.6988825376653836 ) ) ;
#33380=CARTESIAN_POINT ( 'NONE',  ( -70.45090325930956965, -277.6680584775729130, -335.4209417799377206 ) ) ;
#33381=CARTESIAN_POINT ( 'NONE',  ( 28.47094693764329065, -286.7485531986419574, -309.3738563898477310 ) ) ;
#33382=CARTESIAN_POINT ( 'NONE',  ( -95.40437605516592612, -275.2068316463672772, -222.8676421767180784 ) ) ;
#33384=CARTESIAN_POINT ( 'NONE',  ( -97.48747332662306064, -289.1699959026884699, -312.0375157240142130 ) ) ;
#33385=CARTESIAN_POINT ( 'NONE',  ( -67.14189056295913360, -285.0201669947567780, -199.4720395797210131 ) ) ;
#33386=CARTESIAN_POINT ( 'NONE',  ( 16.54851465548530598, -280.5131106840119060, -321.1678506186041204 ) ) ;
#33387=CARTESIAN_POINT ( 'NONE',  ( 20.63405929242779635, -280.7606380779271831, -315.6842493682204918 ) ) ;
#33388=CARTESIAN_POINT ( 'NONE',  ( -111.7594320552299365, -282.5890778349499897, -273.6783914448520250 ) ) ;
#33389=CARTESIAN_POINT ( 'NONE',  ( -105.0620966317721212, -286.9778760011843701, -238.0091167032872477 ) ) ;
#33390=CARTESIAN_POINT ( 'NONE',  ( -104.6293047673641752, -279.3636455854335736, -299.8057892693868780 ) ) ;
#33392=CARTESIAN_POINT ( 'NONE',  ( -37.80881650887317136, -294.0464577399726522, -195.3625682920283566 ) ) ;
#33393=CARTESIAN_POINT ( 'NONE',  ( -73.63287179526206216, -275.7668267350696851, -337.1361288332239496 ) ) ;
#33394=CARTESIAN_POINT ( 'NONE',  ( 13.80857113568835892, -276.9634322458376232, -322.6575034100913513 ) ) ;
#33395=CARTESIAN_POINT ( 'NONE',  ( -6.191466573511966942, -284.6439699244017447, -338.7693878016455642 ) ) ;
#33397=CARTESIAN_POINT ( 'NONE',  ( -64.89862952135668195, -291.3293071720496528, -340.7721363757398763 ) ) ;
#33398=CARTESIAN_POINT ( 'NONE',  ( -47.84812007477871987, -293.1854730478466422, -344.6730768276890444 ) ) ;
#33399=CARTESIAN_POINT ( 'NONE',  ( -3.551126185268555613, -285.6839846275381092, -201.3367944710279858 ) ) ;
#33400=CARTESIAN_POINT ( 'NONE',  ( -104.2733998130901369, -289.3671544889607503, -239.2711197468755699 ) ) ;
#33402=CARTESIAN_POINT ( 'NONE',  ( 35.33180851054449079, -274.0924413248309293, -259.3307870670092825 ) ) ;
#33403=CARTESIAN_POINT ( 'NONE',  ( -70.29330015517498964, -293.6307662981492967, -336.8822239513026489 ) ) ;
#33406=CARTESIAN_POINT ( 'NONE',  ( -83.82849895517507832, -289.9071598957123683, -209.7826744868514481 ) ) ;
#33407=CARTESIAN_POINT ( 'NONE',  ( -109.4509030911634113, -286.3580056145656840, -254.5952550540395691 ) ) ;
#33408=CARTESIAN_POINT ( 'NONE',  ( -59.75011279072997183, -287.5784065720295644, -342.9685353296794119 ) ) ;
#33409=CARTESIAN_POINT ( 'NONE',  ( -110.0058226546812534, -286.1306901084002448, -258.6493158258560925 ) ) ;
#33411=CARTESIAN_POINT ( 'NONE',  ( -27.82564950983397978, -286.9789246063949690, -197.8211530850211375 ) ) ;
#33412=CARTESIAN_POINT ( 'NONE',  ( 30.75471345333757611, -295.9559806990986317, -302.7517930220674316 ) ) ;
#33413=CARTESIAN_POINT ( 'NONE',  ( -111.6539567952122383, -276.4568111293946231, -284.1072218640710503 ) ) ;
#33414=CARTESIAN_POINT ( 'NONE',  ( -14.59189161570405879, -277.0985558225172554, -343.9573297104967082 ) ) ;
#33415=CARTESIAN_POINT ( 'NONE',  ( 18.37075984491076497, -290.9243867938927224, -219.3176462902255537 ) ) ;
#33416=CARTESIAN_POINT ( 'NONE',  ( -72.88608535875843586, -297.5053259332333937, -336.0144408177023365 ) ) ;
#33419=CARTESIAN_POINT ( 'NONE',  ( -41.33307833562736278, -284.6857060914168756, -196.9638474514909490 ) ) ;
#33420=CARTESIAN_POINT ( 'NONE',  ( -83.79789167289104057, -275.8368963041938287, -328.3296919027622494 ) ) ;
#33421=CARTESIAN_POINT ( 'NONE',  ( 37.42014773041214681, -279.4753064729031280, -264.3889532623327341 ) ) ;
#33422=CARTESIAN_POINT ( 'NONE',  ( 26.36249097817102438, -273.4746662289535379, -228.3553589978261016 ) ) ;
#33423=CARTESIAN_POINT ( 'NONE',  ( -109.5940716521211158, -277.7543482192563715, -281.4736099366369331 ) ) ;
#33424=CARTESIAN_POINT ( 'NONE',  ( 35.98316140142789266, -294.9696724109267052, -262.5089811743219457 ) ) ;
#33425=CARTESIAN_POINT ( 'NONE',  ( 29.02598759336025225, -279.9707319588878249, -231.9316691758452293 ) ) ;
#33426=CARTESIAN_POINT ( 'NONE',  ( -66.13464146498840535, -296.3797774291025462, -337.6988858231425752 ) ) ;
#33427=CARTESIAN_POINT ( 'NONE',  ( -36.56380722448715659, -299.3768667954376497, -193.8540952940258251 ) ) ;
#33428=CARTESIAN_POINT ( 'NONE',  ( -81.94243939126651810, -297.2584655173567967, -212.5062755757392665 ) ) ;
#33429=CARTESIAN_POINT ( 'NONE',  ( -33.42888667534835889, -294.1015478314944858, -195.4504159624086412 ) ) ;
#33430=CARTESIAN_POINT ( 'NONE',  ( -23.78799208008210186, -286.3872846946402433, -194.5091640045761778 ) ) ;
#33431=CARTESIAN_POINT ( 'NONE',  ( 36.96621835176514281, -273.8796806781463715, -285.1475554983709344 ) ) ;
#33432=CARTESIAN_POINT ( 'NONE',  ( 23.28614635133079247, -288.0201669887010212, -317.8509082516174544 ) ) ;
#33433=CARTESIAN_POINT ( 'NONE',  ( -110.5043173665690830, -280.7238243642296993, -255.4955348153288242 ) ) ;
#33434=CARTESIAN_POINT ( 'NONE',  ( 32.50159205227141967, -286.3193089501468762, -248.2890646920061499 ) ) ;
#33435=CARTESIAN_POINT ( 'NONE',  ( -111.1692149113089130, -288.3814470610126364, -283.6435902144257284 ) ) ;
#33438=CARTESIAN_POINT ( 'NONE',  ( 3.643948319138460956, -287.9921339471291617, -330.9048860672280057 ) ) ;
#33440=CARTESIAN_POINT ( 'NONE',  ( -111.4970665104632133, -285.7448970575715634, -250.3167702164104185 ) ) ;
#33441=CARTESIAN_POINT ( 'NONE',  ( -108.5845629321353982, -289.2469886099032124, -298.9491349106299367 ) ) ;
#33442=CARTESIAN_POINT ( 'NONE',  ( 38.48421450496085328, -283.2540423829130418, -278.4135232348953082 ) ) ;
#33443=CARTESIAN_POINT ( 'NONE',  ( -42.41418810748496071, -281.3046040939788668, -194.0226077879337083 ) ) ;
#33444=CARTESIAN_POINT ( 'NONE',  ( 33.11413949807556634, -281.1325359539231385, -251.2089778662260358 ) ) ;
#33445=CARTESIAN_POINT ( 'NONE',  ( 34.77629713433318415, -277.2851623698398953, -249.5846316465301413 ) ) ;
#33446=CARTESIAN_POINT ( 'NONE',  ( -13.78204409039318001, -294.7546166827933121, -343.6682977631642188 ) ) ;
#33447=CARTESIAN_POINT ( 'NONE',  ( -93.66913903925652107, -287.8886563336205882, -319.4186595398954864 ) ) ;
#33448=EDGE_CURVE ( 'NONE', #38700, #93199, #74701, .T. ) ;
#33449=CARTESIAN_POINT ( 'NONE',  ( -105.7809614688212037, -271.7011620353396211, -243.7031169602172156 ) ) ;
#33452=CARTESIAN_POINT ( 'NONE',  ( -98.70580278528265694, -285.8959690187934370, -312.5906964755948820 ) ) ;
#33453=CARTESIAN_POINT ( 'NONE',  ( 36.07778864208916758, -294.9131285602464914, -292.7012493243549898 ) ) ;
#33454=CARTESIAN_POINT ( 'NONE',  ( -21.35785909716079800, -283.4932570154115865, -341.7462929848896920 ) ) ;
#33455=CARTESIAN_POINT ( 'NONE',  ( -1.587978628988057528, -275.6486949334394012, -338.2911673900875371 ) ) ;
#33456=CARTESIAN_POINT ( 'NONE',  ( -114.2670865423148143, -291.2285534235827527, -268.3656461346440665 ) ) ;
#33457=CARTESIAN_POINT ( 'NONE',  ( -113.1202429249092631, -282.6609183111559105, -272.7856826508978543 ) ) ;
#33458=CARTESIAN_POINT ( 'NONE',  ( 26.47299462915980683, -293.3169465550612927, -227.2158876293997878 ) ) ;
#33459=CARTESIAN_POINT ( 'NONE',  ( -101.6597603038106712, -290.4128301107849097, -305.0410555933581804 ) ) ;
#33462=CARTESIAN_POINT ( 'NONE',  ( -21.17153989118013158, -109.2489533316710464, -359.0337785304685667 ) ) ;
#33463=CARTESIAN_POINT ( 'NONE',  ( -64.98282404026691950, -284.9268695719707125, -341.4995623601482748 ) ) ;
#33464=CARTESIAN_POINT ( 'NONE',  ( -4.829096099716524648, -292.1237833571632905, -337.9475929042657754 ) ) ;
#33466=CARTESIAN_POINT ( 'NONE',  ( 35.99694277239871099, -280.4492057680265020, -268.5897685596444262 ) ) ;
#33467=CARTESIAN_POINT ( 'NONE',  ( 30.52242004692138622, -275.6898842619803531, -306.8082895407610522 ) ) ;
#33468=CARTESIAN_POINT ( 'NONE',  ( -95.37810012770053447, -281.2045895927852825, -223.1191376488047240 ) ) ;
#33469=CARTESIAN_POINT ( 'NONE',  ( -45.93041767256378449, -156.1281930031302068, -363.3478848798407626 ) ) ;
#33470=CARTESIAN_POINT ( 'NONE',  ( 10.46857768926897592, -279.2719313653462336, -210.6880551476552625 ) ) ;
#33471=CARTESIAN_POINT ( 'NONE',  ( -112.0365078248271260, -282.5653471247208586, -270.8964869736045102 ) ) ;
#33472=CARTESIAN_POINT ( 'NONE',  ( -95.99516178219309381, -275.0671097645934537, -222.3817486476455372 ) ) ;
#33473=CARTESIAN_POINT ( 'NONE',  ( -88.54050398348223894, -296.2860443105471973, -322.5539042674809593 ) ) ;
#33475=CARTESIAN_POINT ( 'NONE',  ( -100.1242550243702709, -289.7596351732216817, -232.1564811165874573 ) ) ;
#33476=CARTESIAN_POINT ( 'NONE',  ( -9.241333025187392636, -277.3456664461765513, -341.9410184804669370 ) ) ;
#33477=CARTESIAN_POINT ( 'NONE',  ( -5.308056246438822789, -274.4858272961020589, -204.7512142507426347 ) ) ;
#33478=CARTESIAN_POINT ( 'NONE',  ( 35.44097946285869938, -274.1651124572006779, -246.0239343167204140 ) ) ;
#33480=CARTESIAN_POINT ( 'NONE',  ( -111.5704608358709891, -270.6942485587154579, -259.2817424984529566 ) ) ;
#33484=CARTESIAN_POINT ( 'NONE',  ( 35.65880787313304268, -282.5365407540246565, -263.1071437057715912 ) ) ;
#33485=CARTESIAN_POINT ( 'NONE',  ( 25.11044511923328670, -283.8919668631231161, -313.6703089757065186 ) ) ;
#33486=CARTESIAN_POINT ( 'NONE',  ( -108.8214824896591892, -283.6982118289224104, -285.7350846272551053 ) ) ;
#33487=CARTESIAN_POINT ( 'NONE',  ( 21.46215340906459446, -274.5719250932676232, -314.9542477927584514 ) ) ;
#33488=CARTESIAN_POINT ( 'NONE',  ( 36.92249123114469000, -283.3888200197109768, -268.5298594868648934 ) ) ;
#33489=CARTESIAN_POINT ( 'NONE',  ( -32.39315626288333050, -275.4686443762308272, -343.9385588584381708 ) ) ;
#33491=CARTESIAN_POINT ( 'NONE',  ( 35.95166978979703032, -276.6118735473925767, -268.8419080778610919 ) ) ;
#33493=CARTESIAN_POINT ( 'NONE',  ( -59.26586970594906489, -280.5781960372398771, -196.7167725893437762 ) ) ;
#33496=CARTESIAN_POINT ( 'NONE',  ( -36.60168210301413438, -287.9217569565474832, -194.5870990019050168 ) ) ;
#33497=CARTESIAN_POINT ( 'NONE',  ( -42.41109624394971434, -294.3148843736417462, -343.3467532140356298 ) ) ;
#33499=CARTESIAN_POINT ( 'NONE',  ( -100.6014699525223079, -289.3225988504343036, -314.0819860938323700 ) ) ;
#33500=CARTESIAN_POINT ( 'NONE',  ( 22.82830041259893150, -285.1968662942176138, -227.1754310312921916 ) ) ;
#33501=CARTESIAN_POINT ( 'NONE',  ( -11.80059340024893899, -284.9660469232246669, -201.3464327038570900 ) ) ;
#33502=CARTESIAN_POINT ( 'NONE',  ( -92.41235757496139058, -289.4902427952504240, -220.8932383347653570 ) ) ;
#33503=CARTESIAN_POINT ( 'NONE',  ( -105.5774482385071451, -285.3958661654552316, -297.5366490133638422 ) ) ;
#33504=CARTESIAN_POINT ( 'NONE',  ( 17.42490343750725046, -274.2695623518728212, -321.6019199178481358 ) ) ;
#33506=CARTESIAN_POINT ( 'NONE',  ( -30.93063966012798360, -284.5317392400209542, -194.4181336177512378 ) ) ;
#33507=CARTESIAN_POINT ( 'NONE',  ( -40.38528535353915316, -300.0141807748269116, -195.3721238207088504 ) ) ;
#33508=CARTESIAN_POINT ( 'NONE',  ( 20.96647093977610510, -286.2041736542307149, -317.8174870631714839 ) ) ;
#33509=CARTESIAN_POINT ( 'NONE',  ( -43.78369384797323249, -280.9101416243232165, -197.3593056544557669 ) ) ;
#33510=CARTESIAN_POINT ( 'NONE',  ( -31.93265467183951856, -290.9843433520939584, -345.3842212363069279 ) ) ;
#33513=CARTESIAN_POINT ( 'NONE',  ( -91.64479744948833684, -297.7387546211278391, -322.9014626598053042 ) ) ;
#33515=CARTESIAN_POINT ( 'NONE',  ( -46.68092246048014005, -277.9335628596838319, -195.8923586338238181 ) ) ;
#33516=CARTESIAN_POINT ( 'NONE',  ( 34.31595104981452948, -292.3955499653098400, -242.4770524530541138 ) ) ;
#33517=CARTESIAN_POINT ( 'NONE',  ( -105.4932675079784872, -295.3276378690839010, -242.0449692854151920 ) ) ;
#33518=CARTESIAN_POINT ( 'NONE',  ( 33.93795780632670755, -280.0017083555510453, -252.4087159367159927 ) ) ;
#33519=CARTESIAN_POINT ( 'NONE',  ( 34.91269352859074360, -273.4002870889214591, -252.4553424217140787 ) ) ;
#33520=CARTESIAN_POINT ( 'NONE',  ( 31.28293176319303015, -294.5183756526157595, -244.0570617375843199 ) ) ;
#33521=CARTESIAN_POINT ( 'NONE',  ( -69.91165696735023971, -300.1233781216987495, -202.8022627189028810 ) ) ;
#33522=CARTESIAN_POINT ( 'NONE',  ( -102.5333889694384197, -294.5095055384285843, -310.0190485595027212 ) ) ;
#33523=CARTESIAN_POINT ( 'NONE',  ( -30.70211858851053321, -293.2091590906264287, -346.0571546714827491 ) ) ;
#33524=CARTESIAN_POINT ( 'NONE',  ( -94.76198562876894016, -292.6228495563988190, -224.3162502132267946 ) ) ;
#33526=CARTESIAN_POINT ( 'NONE',  ( -98.44001350465183009, -291.9129763238455553, -230.0248489907159239 ) ) ;
#33528=CARTESIAN_POINT ( 'NONE',  ( -100.0643908004630305, -282.0095242350653280, -312.2192592017375432 ) ) ;
#33529=CARTESIAN_POINT ( 'NONE',  ( 35.64194322172812690, -293.5934137414293446, -273.4889707359823774 ) ) ;
#33530=CARTESIAN_POINT ( 'NONE',  ( 10.82300856513808363, -280.6969743179029706, -210.2164851128124212 ) ) ;
#33531=CARTESIAN_POINT ( 'NONE',  ( -101.4039048203670745, -283.6558696384626046, -313.1390636979091937 ) ) ;
#33532=CARTESIAN_POINT ( 'NONE',  ( -85.89337988077159025, -287.7258796903413440, -327.3747957183749691 ) ) ;
#33533=CARTESIAN_POINT ( 'NONE',  ( -96.92711670422742998, -282.0810474347836134, -314.6380150509479563 ) ) ;
#33535=CARTESIAN_POINT ( 'NONE',  ( -50.79817612958569129, -278.3631099662396196, -195.2503264498887461 ) ) ;
#33536=CARTESIAN_POINT ( 'NONE',  ( 35.55951303419863763, -286.1698025707267448, -246.3814091679362548 ) ) ;
#33538=CARTESIAN_POINT ( 'NONE',  ( 26.49475910102298570, -295.6548031923206281, -307.3928190887405094 ) ) ;
#33539=CARTESIAN_POINT ( 'NONE',  ( 22.19342012054821467, -277.6244730557907587, -318.2793755749885349 ) ) ;
#33540=CARTESIAN_POINT ( 'NONE',  ( -87.11304259547296169, -277.4355641407343001, -323.7923911819154910 ) ) ;
#33541=CARTESIAN_POINT ( 'NONE',  ( -58.94071754505114313, -291.9468757793724194, -196.4525092071985739 ) ) ;
#33542=CARTESIAN_POINT ( 'NONE',  ( -35.95069252803639870, -281.1147194441184638, -345.9211890928669959 ) ) ;
#33543=CARTESIAN_POINT ( 'NONE',  ( 34.94812936448611396, -292.4556254315568822, -258.5527877890277750 ) ) ;
#33544=CARTESIAN_POINT ( 'NONE',  ( -105.3634549566303207, -294.1369017799314065, -301.9529130517282738 ) ) ;
#33547=CARTESIAN_POINT ( 'NONE',  ( 3.845913698009563841, -293.9884226659847855, -330.7065313031921505 ) ) ;
#33549=CARTESIAN_POINT ( 'NONE',  ( -105.5795714935544112, -288.2666405000203440, -254.7536222014695397 ) ) ;
#33550=CARTESIAN_POINT ( 'NONE',  ( -60.06696186555931405, -296.8235170907243514, -196.9819479541712610 ) ) ;
#33551=CARTESIAN_POINT ( 'NONE',  ( 37.44471777992286121, -279.8470267678326877, -282.5786095512858651 ) ) ;
#33552=CARTESIAN_POINT ( 'NONE',  ( 24.29596346786136962, -288.2613957561225106, -225.0389743856972871 ) ) ;
#33553=CARTESIAN_POINT ( 'NONE',  ( -37.27014957742278511, -288.8845514035576230, -343.3610829487153069 ) ) ;
#33554=CARTESIAN_POINT ( 'NONE',  ( -107.7735877262127531, -279.7857744234878510, -292.2126405768848372 ) ) ;
#33555=CARTESIAN_POINT ( 'NONE',  ( -109.5673363045812181, -294.3282902113879800, -289.2612382266176496 ) ) ;
#33556=CARTESIAN_POINT ( 'NONE',  ( -103.6664114205074299, -297.8717295870629300, -303.3251021515311550 ) ) ;
#33557=CARTESIAN_POINT ( 'NONE',  ( -97.98551098742142074, -276.7749808841734307, -311.7067188312922212 ) ) ;
#33559=CARTESIAN_POINT ( 'NONE',  ( -65.53030855817522138, -297.3603538583422505, -198.6721232773958832 ) ) ;
#33560=CARTESIAN_POINT ( 'NONE',  ( -70.59414612453876714, -291.4142152710654727, -336.9754656033932747 ) ) ;
#33561=CARTESIAN_POINT ( 'NONE',  ( 28.77132586717855034, -294.6548244913639678, -232.4730168480541010 ) ) ;
#33564=CARTESIAN_POINT ( 'NONE',  ( 1.372587174990538506, -289.1712858943852780, -332.3699611157591676 ) ) ;
#33567=CARTESIAN_POINT ( 'NONE',  ( -113.1019969162496892, -297.0347547378974582, -283.8409921459889915 ) ) ;
#33568=CARTESIAN_POINT ( 'NONE',  ( -111.6610807558444094, -288.5036978710386961, -285.1556981684919947 ) ) ;
#33569=CARTESIAN_POINT ( 'NONE',  ( -73.27453619583678801, -297.9225736999538299, -202.2245691154867302 ) ) ;
#33574=CARTESIAN_POINT ( 'NONE',  ( 21.87941867036990828, -289.7238863253596151, -318.5020260311712832 ) ) ;
#33575=CARTESIAN_POINT ( 'NONE',  ( -88.52914483777347243, -275.9090924074130271, -206.2264541496106460 ) ) ;
#33576=CARTESIAN_POINT ( 'NONE',  ( 38.15619258392178637, -280.7178121307047718, -255.7535520339510526 ) ) ;
#33577=CARTESIAN_POINT ( 'NONE',  ( -103.8798540636037586, -287.0064152887067053, -236.1163739430591875 ) ) ;
#33578=CARTESIAN_POINT ( 'NONE',  ( -23.87180051405622905, -284.7955885954241921, -195.0931656201879605 ) ) ;
#33579=CARTESIAN_POINT ( 'NONE',  ( -49.13997931962696697, -271.9014379775259727, -196.4112388732575596 ) ) ;
#33580=CARTESIAN_POINT ( 'NONE',  ( -51.86589950027864404, -275.7851653991967851, -197.2989762936699663 ) ) ;
#33582=CARTESIAN_POINT ( 'NONE',  ( -92.72854861731995868, -289.3302557942081989, -220.6066478652665523 ) ) ;
#33583=CARTESIAN_POINT ( 'NONE',  ( -113.1425260752796902, -280.4326150102098723, -268.7839863158469029 ) ) ;
#33585=CARTESIAN_POINT ( 'NONE',  ( 2.703984594086757731, -280.6055182956760063, -209.2648739963373998 ) ) ;
#33586=CARTESIAN_POINT ( 'NONE',  ( 20.60180239076771258, -280.2741367026085300, -225.7712379358224268 ) ) ;
#33587=CARTESIAN_POINT ( 'NONE',  ( 34.91438619334918059, -276.9592642898892905, -296.2189058253874805 ) ) ;
#33588=CARTESIAN_POINT ( 'NONE',  ( 30.37800443713192777, -279.8810531732180493, -234.4422591463007564 ) ) ;
#33589=CARTESIAN_POINT ( 'NONE',  ( -109.6225879400218872, -263.9640009610400853, -305.6697541383538237 ) ) ;
#33590=CARTESIAN_POINT ( 'NONE',  ( 36.35656919146170196, -276.2210926640910884, -248.6955815581138154 ) ) ;
#33592=CARTESIAN_POINT ( 'NONE',  ( -34.80219443597819406, -299.5086240258658563, -193.9497409019863028 ) ) ;
#33593=EDGE_CURVE ( 'NONE', #9910, #64985, #55100, .T. ) ;
#33594=CARTESIAN_POINT ( 'NONE',  ( -4.771743288812468897, -285.1233781216987495, -337.9199732462171255 ) ) ;
#33596=DIRECTION ( 'NONE',  ( 0.000000000000000000, 0.000000000000000000, 1.000000000000000000 ) ) ;
#33597=CARTESIAN_POINT ( 'NONE',  ( 3.799404484734379306, -289.5638994157276329, -331.0988193956028454 ) ) ;
#33598=CARTESIAN_POINT ( 'NONE',  ( 20.72929455207008331, -289.9812843131265936, -319.3686030540673642 ) ) ;
#33599=CARTESIAN_POINT ( 'NONE',  ( -70.02547447582276163, -288.8430648307809747, -335.7635557315431925 ) ) ;
#33600=CARTESIAN_POINT ( 'NONE',  ( -40.80741904840011358, -285.5174441916616388, -193.4486014770332929 ) ) ;
#33601=CARTESIAN_POINT ( 'NONE',  ( -76.76918040625621131, -209.2117619618190929, -357.1497412455196354 ) ) ;
#33602=CARTESIAN_POINT ( 'NONE',  ( 35.93156225681961757, -280.0722878596320129, -279.5781497160837148 ) ) ;
#33603=CARTESIAN_POINT ( 'NONE',  ( 36.68558903127784276, -289.4930043250041649, -276.5613092504442534 ) ) ;
#33604=CARTESIAN_POINT ( 'NONE',  ( 18.11395929613510347, -280.7180154664252427, -318.8933504824460101 ) ) ;
#33605=CARTESIAN_POINT ( 'NONE',  ( -71.18355912115484330, -280.9108686451132826, -205.1091223539073098 ) ) ;
#33606=CARTESIAN_POINT ( 'NONE',  ( -8.708786258203033981, -277.1594643278485819, -337.5918182459787431 ) ) ;
#33607=CARTESIAN_POINT ( 'NONE',  ( -103.4634812553831864, -288.8399084798168133, -309.1431809583249333 ) ) ;
#33608=CARTESIAN_POINT ( 'NONE',  ( -91.79577878998694018, -286.1021707033149823, -216.1493836683731047 ) ) ;
#33609=CARTESIAN_POINT ( 'NONE',  ( -111.6634124857076245, -285.2960648011215312, -250.2658429835092306 ) ) ;
#33610=CARTESIAN_POINT ( 'NONE',  ( 33.94087426313222977, -281.9264890973526008, -286.1026106912966043 ) ) ;
#33611=VERTEX_POINT ( 'NONE', #91842 ) ;
#33613=CARTESIAN_POINT ( 'NONE',  ( -104.0569247897468443, -291.9407146101873423, -306.2691153697310824 ) ) ;
#33615=CARTESIAN_POINT ( 'NONE',  ( 6.229211675588853581, -291.3150797694533480, -207.4733296905254178 ) ) ;
#33616=CARTESIAN_POINT ( 'NONE',  ( 33.12097590376699685, -274.8744770714257015, -290.3674372353284525 ) ) ;
#33618=CARTESIAN_POINT ( 'NONE',  ( -93.62053362882431884, -295.1853100060159250, -322.7828581877265606 ) ) ;
#33619=CARTESIAN_POINT ( 'NONE',  ( -49.78694387216549444, -290.3705441428924132, -197.6744412394347421 ) ) ;
#33620=CARTESIAN_POINT ( 'NONE',  ( -42.48217194291863308, -293.3577302635454203, -344.1957275069991624 ) ) ;
#33621=CARTESIAN_POINT ( 'NONE',  ( -88.92930951457302058, -291.0021749139226586, -322.5707824346350776 ) ) ;
#33623=CARTESIAN_POINT ( 'NONE',  ( -93.93204246742143937, -291.8692315442620497, -319.5803602048571292 ) ) ;
#33624=CARTESIAN_POINT ( 'NONE',  ( 35.31769813155879234, -291.7988961752489558, -289.6131379771490515 ) ) ;
#33625=CARTESIAN_POINT ( 'NONE',  ( 4.835301026201904051, -296.4830329575373185, -332.4397731466709729 ) ) ;
#33626=CARTESIAN_POINT ( 'NONE',  ( -73.68277161649744755, -286.4983424837704433, -206.7640687634293499 ) ) ;
#33627=CARTESIAN_POINT ( 'NONE',  ( 36.00084614671346372, -295.7639170392411074, -286.8783198665047962 ) ) ;
#33628=CARTESIAN_POINT ( 'NONE',  ( 31.04944341120724616, -277.1169673663370645, -238.5974423883914994 ) ) ;
#33629=CARTESIAN_POINT ( 'NONE',  ( 25.73116992351905807, -274.9250401541016231, -313.9249831452214039 ) ) ;
#33630=CARTESIAN_POINT ( 'NONE',  ( -23.38597822280161154, -297.4198807086748957, -193.5244381569562506 ) ) ;
#33631=CARTESIAN_POINT ( 'NONE',  ( 8.186328144667884388, -274.6599255679947760, -328.7802653937671380 ) ) ;
#33632=CARTESIAN_POINT ( 'NONE',  ( -97.55640773327610304, -277.2327012847827632, -226.5946560763432558 ) ) ;
#33633=CARTESIAN_POINT ( 'NONE',  ( 52.40925428718954748, -300.5139553254558109, -196.8474091074338332 ) ) ;
#33635=CARTESIAN_POINT ( 'NONE',  ( -86.87328784996806519, -297.1830022178324384, -324.7853472705846798 ) ) ;
#33637=CARTESIAN_POINT ( 'NONE',  ( -97.02036411700407825, -297.9446190521592825, -228.0402154435760451 ) ) ;
#33640=CARTESIAN_POINT ( 'NONE',  ( -69.95063100753816343, -287.4995286371100747, -338.3095616981197509 ) ) ;
#33641=CARTESIAN_POINT ( 'NONE',  ( -104.3788646822989108, -272.7753129095747227, -241.3363363248622591 ) ) ;
#33642=CARTESIAN_POINT ( 'NONE',  ( 12.07757810788665331, -286.7172453998858828, -211.2429610981553765 ) ) ;
#33643=CARTESIAN_POINT ( 'NONE',  ( -5.639080900124533891, -288.3132061691605941, -340.5087353740714775 ) ) ;
#33644=CARTESIAN_POINT ( 'NONE',  ( -106.2787521760149048, -298.9302509307642595, -239.8002878759974692 ) ) ;
#33645=CARTESIAN_POINT ( 'NONE',  ( 35.21759690324666536, -291.7876982258098337, -288.6689535812006397 ) ) ;
#33647=CARTESIAN_POINT ( 'NONE',  ( 23.26922539889932651, -281.3818258528739307, -317.6102767978092061 ) ) ;
#33650=CARTESIAN_POINT ( 'NONE',  ( 18.85470292168867346, -278.8607530831927193, -220.6167120060577815 ) ) ;
#33652=CARTESIAN_POINT ( 'NONE',  ( -34.57834259461453996, -287.8117194252216109, -343.7560065552784181 ) ) ;
#33654=CARTESIAN_POINT ( 'NONE',  ( -92.06913834561316889, -287.8330834980292821, -321.7196185466897873 ) ) ;
#33655=CARTESIAN_POINT ( 'NONE',  ( -37.16796817485462157, -299.6545001417760545, -196.5581842902400069 ) ) ;
#33656=CARTESIAN_POINT ( 'NONE',  ( 23.79466047301081844, -283.5921448908923139, -316.1972577293420841 ) ) ;
#33657=CARTESIAN_POINT ( 'NONE',  ( -29.25402909278367503, -296.1730293061041266, -195.0086224598954061 ) ) ;
#33658=CARTESIAN_POINT ( 'NONE',  ( -38.88507961700194215, -283.0720126773367724, -343.3572918297165302 ) ) ;
#33659=CARTESIAN_POINT ( 'NONE',  ( 7.677174245882701697, -276.1059256043942582, -212.1487836749950588 ) ) ;
#33660=CARTESIAN_POINT ( 'NONE',  ( 35.38546615758858849, -283.3169278407723368, -252.0373646458685073 ) ) ;
#33661=CARTESIAN_POINT ( 'NONE',  ( -105.6995143030591322, -271.8265461743915239, -243.7365338049869763 ) ) ;
#33663=CARTESIAN_POINT ( 'NONE',  ( 204.9607212768056002, 294.2270030158686609, -54.00000000002630429 ) ) ;
#33664=CARTESIAN_POINT ( 'NONE',  ( 36.28760096717648764, -293.1025409726746602, -247.8283413065005334 ) ) ;
#33665=CARTESIAN_POINT ( 'NONE',  ( -82.49308156484593724, -287.4118975820412061, -210.9203949553242126 ) ) ;
#33667=CARTESIAN_POINT ( 'NONE',  ( -19.11405058567864046, -280.3380690714490129, -350.3683826091709648 ) ) ;
#33668=CARTESIAN_POINT ( 'NONE',  ( -38.55268814232832852, -276.2641467717829755, -347.1900990328595071 ) ) ;
#33669=CARTESIAN_POINT ( 'NONE',  ( -70.31157119121917276, -287.8792309234474942, -339.0735480313547896 ) ) ;
#33670=CARTESIAN_POINT ( 'NONE',  ( -83.21129710071788566, -285.2133120241918505, -328.1040309522289817 ) ) ;
#33671=CARTESIAN_POINT ( 'NONE',  ( -72.11066116754413713, -279.2786817679706246, -335.7137108542152646 ) ) ;
#33673=CARTESIAN_POINT ( 'NONE',  ( -111.7897729462377185, -286.1942796256317934, -253.1538303024127856 ) ) ;
#33674=CARTESIAN_POINT ( 'NONE',  ( -37.55701601160195935, -281.8498643805666006, -343.7703736456794559 ) ) ;
#33675=CARTESIAN_POINT ( 'NONE',  ( -69.40069153408602176, -281.6304327578977791, -202.5583029722567403 ) ) ;
#33676=CARTESIAN_POINT ( 'NONE',  ( 24.47860339448041245, -275.1084676483693556, -224.4563243668394819 ) ) ;
#33677=CARTESIAN_POINT ( 'NONE',  ( -56.92607864134298268, -277.1311549983469149, -344.8839635698042798 ) ) ;
#33678=CARTESIAN_POINT ( 'NONE',  ( -4.892113991333567391, -296.5416556103949688, -337.3702674550272604 ) ) ;
#33680=ADVANCED_FACE ( 'NONE', ( #20372 ), #91103, .T. ) ;
#33682=CARTESIAN_POINT ( 'NONE',  ( -111.3881803080732311, -294.8963911817058374, -254.2562071646758284 ) ) ;
#33683=CARTESIAN_POINT ( 'NONE',  ( 32.92093513569110286, -274.7930572003534735, -250.1515436607077447 ) ) ;
#33684=CARTESIAN_POINT ( 'NONE',  ( -62.75562827202377036, -298.8085967473858204, -198.0035007908743410 ) ) ;
#33685=CARTESIAN_POINT ( 'NONE',  ( 15.74086640570477158, -288.5767274524653203, -218.7838444669939975 ) ) ;
#33686=CARTESIAN_POINT ( 'NONE',  ( 6.234087937547879044, -295.9928573833530550, -333.0662213700896928 ) ) ;
#33687=CARTESIAN_POINT ( 'NONE',  ( 0.3585246579834400760, -295.7666134188271485, -337.0598152207402336 ) ) ;
#33688=CARTESIAN_POINT ( 'NONE',  ( -93.77798925993877788, -291.8680659363610630, -319.5809047017456237 ) ) ;
#33689=CARTESIAN_POINT ( 'NONE',  ( -49.41317454312584800, -277.8977340672214495, -196.5078314649684899 ) ) ;
#33690=CARTESIAN_POINT ( 'NONE',  ( -108.4857575370526064, -280.1857419737564783, -292.4387241674479014 ) ) ;
#33691=CARTESIAN_POINT ( 'NONE',  ( -109.8747436432718700, -294.8485742719273048, -253.6197978293804454 ) ) ;
#33692=CARTESIAN_POINT ( 'NONE',  ( -16.45917374120841004, -284.6456546521537234, -343.2456369855314051 ) ) ;
#33693=CARTESIAN_POINT ( 'NONE',  ( 32.13792627948375014, -286.1631519168715840, -246.9772006941156519 ) ) ;
#33694=CARTESIAN_POINT ( 'NONE',  ( -111.5752165548071986, -274.2545102287181180, -284.0995610720992772 ) ) ;
#33696=CARTESIAN_POINT ( 'NONE',  ( -108.6846531153470607, -284.4249090364280050, -254.7377143622873064 ) ) ;
#33698=CARTESIAN_POINT ( 'NONE',  ( 34.30365023913424238, -282.9795592934676165, -297.7186814684547471 ) ) ;
#33699=VECTOR ( 'NONE', #35523, 999.9999999999998863 ) ;
#33700=CARTESIAN_POINT ( 'NONE',  ( -92.03681255600260158, -273.5764303066907246, -221.9820712441353692 ) ) ;
#33701=CARTESIAN_POINT ( 'NONE',  ( -52.08176782460245846, -284.6625701657092122, -195.1356122146114842 ) ) ;
#33702=CARTESIAN_POINT ( 'NONE',  ( -33.93773580570187676, -281.0352421516735717, -193.6719190019195196 ) ) ;
#33703=DIRECTION ( 'NONE',  ( 1.000000000000000000, 0.000000000000000000, 0.000000000000000000 ) ) ;
#33704=CARTESIAN_POINT ( 'NONE',  ( -39.58643605664883580, -281.5445938236794632, -194.0745400995285479 ) ) ;
#33705=CARTESIAN_POINT ( 'NONE',  ( 17.14502302725733784, -281.4556240429934064, -216.0231233488367479 ) ) ;
#33706=CARTESIAN_POINT ( 'NONE',  ( -105.5795714935544112, -288.2666405000203440, -254.7536222014695397 ) ) ;
#33707=CARTESIAN_POINT ( 'NONE',  ( 26.31071593616584181, -23.39576146109087773, -345.1909842725040107 ) ) ;
#33709=CARTESIAN_POINT ( 'NONE',  ( -18.84244262916453394, -276.2909034966050399, -197.7966492087222434 ) ) ;
#33710=CARTESIAN_POINT ( 'NONE',  ( 64.17530680665127818, 48.17049669212057239, -318.6057662566004183 ) ) ;
#33712=CARTESIAN_POINT ( 'NONE',  ( -32.83916367470790476, -278.1292794572481171, -195.8522328115398921 ) ) ;
#33713=CARTESIAN_POINT ( 'NONE',  ( 10.46364476597024584, -294.4615808310846319, -211.2288719802450032 ) ) ;
#33714=CARTESIAN_POINT ( 'NONE',  ( -108.6931708251894690, -295.6912616085022592, -286.2626996000261670 ) ) ;
#33715=CARTESIAN_POINT ( 'NONE',  ( -36.37284023812897260, -291.5716499810744153, -193.4157345928995255 ) ) ;
#33717=AXIS2_PLACEMENT_3D ( 'NONE', #50600, #5652, #20325 ) ;
#33718=CARTESIAN_POINT ( 'NONE',  ( -105.4408738666261058, -294.6758408404045895, -305.1347442407738413 ) ) ;
#33719=CARTESIAN_POINT ( 'NONE',  ( 24.21246393252809170, -285.3922174050144918, -229.5558423132454493 ) ) ;
#33720=CARTESIAN_POINT ( 'NONE',  ( 32.71345683582602959, -295.7356792130172494, -295.0740974668204899 ) ) ;
#33721=CARTESIAN_POINT ( 'NONE',  ( -87.25153948568416240, -285.0801928818528950, -324.3774728692913527 ) ) ;
#33723=CARTESIAN_POINT ( 'NONE',  ( -108.1547181753909257, -291.8715086279845536, -240.7243724226984511 ) ) ;
#33725=CARTESIAN_POINT ( 'NONE',  ( 11.96283158980991068, -282.8366508234660159, -324.2781987046529935 ) ) ;
#33726=CARTESIAN_POINT ( 'NONE',  ( -95.29122354764726310, -294.6668258874401545, -320.4596354743204074 ) ) ;
#33727=CARTESIAN_POINT ( 'NONE',  ( -111.0800873768386339, -291.6265468158190970, -248.7553533214974379 ) ) ;
#33728=CARTESIAN_POINT ( 'NONE',  ( -58.92743026163221742, -292.2724904976134894, -196.5127384628947027 ) ) ;
#33729=CARTESIAN_POINT ( 'NONE',  ( 35.68030624157331943, -287.6917801846342968, -268.3103421497913814 ) ) ;
#33732=CARTESIAN_POINT ( 'NONE',  ( -66.42798308569273047, -297.2893707665758711, -340.3343179143163866 ) ) ;
#33734=CARTESIAN_POINT ( 'NONE',  ( -23.45422380015054742, -296.9074280743311078, -193.8572936979943790 ) ) ;
#33735=CARTESIAN_POINT ( 'NONE',  ( -69.83392783122764058, -278.6721572194342684, -204.7144357722766017 ) ) ;
#33736=CARTESIAN_POINT ( 'NONE',  ( 24.43420870566513869, -274.4495469477350866, -224.4997617970815043 ) ) ;
#33737=CARTESIAN_POINT ( 'NONE',  ( -106.4493367498670295, -295.3717816249535417, -244.6241461178034058 ) ) ;
#33738=CARTESIAN_POINT ( 'NONE',  ( -24.08615795874431598, -278.7416405388045746, -343.4555944186350871 ) ) ;
#33739=CARTESIAN_POINT ( 'NONE',  ( 18.22563593566900764, -272.9994053363270154, -221.0595528862527885 ) ) ;
#33740=CARTESIAN_POINT ( 'NONE',  ( -95.91196825982326857, -297.1389466710945158, -314.6159008857245567 ) ) ;
#33741=CARTESIAN_POINT ( 'NONE',  ( -52.71326549373046788, -298.9303599095174491, -198.6295784983753379 ) ) ;
#33743=CARTESIAN_POINT ( 'NONE',  ( -11.31113936669362374, -296.3188266206519756, -342.0330977658765050 ) ) ;
#33745=CARTESIAN_POINT ( 'NONE',  ( -108.5393859029297943, -270.8902628781388557, -245.6771891607730822 ) ) ;
#33746=CARTESIAN_POINT ( 'NONE',  ( -81.79760104361372441, -292.0800045337432493, -212.2663282159022344 ) ) ;
#33747=CARTESIAN_POINT ( 'NONE',  ( -101.6296669525037117, -289.6138784773024781, -234.4454371296471606 ) ) ;
#33749=CARTESIAN_POINT ( 'NONE',  ( 36.43623797249316709, -276.3190514822618979, -292.2328912709730844 ) ) ;
#33750=CARTESIAN_POINT ( 'NONE',  ( -90.06407026925775483, -297.6149837066819828, -219.7670809749123748 ) ) ;
#33751=CARTESIAN_POINT ( 'NONE',  ( -34.01369287405827180, -282.0737145102760337, -195.0794391186080361 ) ) ;
#33752=CARTESIAN_POINT ( 'NONE',  ( 38.17834042626236624, -280.3921806532635514, -282.6911801347736741 ) ) ;
#33754=CARTESIAN_POINT ( 'NONE',  ( 5.807221992082605588, -275.8324040408410269, -334.0123811767265920 ) ) ;
#33755=CARTESIAN_POINT ( 'NONE',  ( -2.360428848575252925, -281.7739240110116725, -334.6320515182482609 ) ) ;
#33756=CARTESIAN_POINT ( 'NONE',  ( 36.19650027554965988, -279.3518397082912088, -254.7379053054851852 ) ) ;
#33758=CARTESIAN_POINT ( 'NONE',  ( -8.725072674853340260, -273.0086725489012451, -202.5095404288539100 ) ) ;
#33759=CARTESIAN_POINT ( 'NONE',  ( -74.71650625273734647, -279.5493441005215232, -335.4433520056854832 ) ) ;
#33761=FACE_BOUND ( 'NONE', #28526, .T. ) ;
#33762=CARTESIAN_POINT ( 'NONE',  ( -30.57415178395767796, -296.3756381714261465, -194.3764399578238624 ) ) ;
#33763=CARTESIAN_POINT ( 'NONE',  ( 34.74273139890103579, -277.8266213288238191, -291.7106475035720905 ) ) ;
#33764=CARTESIAN_POINT ( 'NONE',  ( -75.26321996967618588, -271.5469468724480748, -205.5942532011225694 ) ) ;
#33766=CARTESIAN_POINT ( 'NONE',  ( -112.7691468501050451, -286.4050046173633746, -275.6419655058780904 ) ) ;
#33769=CARTESIAN_POINT ( 'NONE',  ( -24.34095841460435850, -286.8861492431840361, -344.2776954139054055 ) ) ;
#33771=CARTESIAN_POINT ( 'NONE',  ( 34.15876571452299260, -292.5652325961062274, -286.9939472881684992 ) ) ;
#33772=CARTESIAN_POINT ( 'NONE',  ( 31.10977764642794696, -285.3111224219507562, -241.5005440180586049 ) ) ;
#33773=CARTESIAN_POINT ( 'NONE',  ( -71.74250447947856912, -195.9422791308210492, -360.7315132586310824 ) ) ;
#33774=CARTESIAN_POINT ( 'NONE',  ( -100.1077446438986129, -295.1069028352944770, -229.2132633096373411 ) ) ;
#33775=CARTESIAN_POINT ( 'NONE',  ( -54.78712749521336889, -284.3117141781163468, -196.0754207396757636 ) ) ;
#33776=CARTESIAN_POINT ( 'NONE',  ( -86.02705451083080845, -280.9639830613383538, -214.8978266819527789 ) ) ;
#33777=CARTESIAN_POINT ( 'NONE',  ( 36.40632889669196715, -289.0187437901540193, -291.1272920222765492 ) ) ;
#33778=CARTESIAN_POINT ( 'NONE',  ( 19.01666979615950481, -280.4940768126017474, -321.4057884394308076 ) ) ;
#33779=CARTESIAN_POINT ( 'NONE',  ( -95.76832199553885516, -289.9375932327725991, -314.1464605852987688 ) ) ;
#33781=CARTESIAN_POINT ( 'NONE',  ( -49.25503182952828496, -281.3226153242526948, -197.7426117766690368 ) ) ;
#33782=CARTESIAN_POINT ( 'NONE',  ( 27.92082260691312356, -281.9056627253713145, -237.1821436241081926 ) ) ;
#33783=CARTESIAN_POINT ( 'NONE',  ( 18.42437677322572398, -290.2359783716213428, -321.0612241675873975 ) ) ;
#33784=ORIENTED_EDGE ( 'NONE', *, *, #72569, .T. ) ;
#33786=CARTESIAN_POINT ( 'NONE',  ( -83.58009169530156157, -273.4378093803254046, -208.7231973228109041 ) ) ;
#33787=CARTESIAN_POINT ( 'NONE',  ( -87.82360478376411095, -291.7412389053965853, -325.4168866121209476 ) ) ;
#33788=CARTESIAN_POINT ( 'NONE',  ( -110.4683760289727132, -275.2662352645559167, -253.7030783399848985 ) ) ;
#33790=CARTESIAN_POINT ( 'NONE',  ( 14.77468822335568355, -272.7842003558055808, -216.1955339830585672 ) ) ;
#33791=CARTESIAN_POINT ( 'NONE',  ( 128.9467878515196162, -299.5541904835127980, -195.3611179825600175 ) ) ;
#33792=CARTESIAN_POINT ( 'NONE',  ( -90.17226282765506085, -294.1836238426474210, -325.3461868356761784 ) ) ;
#33793=CARTESIAN_POINT ( 'NONE',  ( -103.7719314678626858, -296.4710905878346807, -239.8253461820677899 ) ) ;
#33795=CARTESIAN_POINT ( 'NONE',  ( 27.65099010683070802, -289.5426114480258093, -305.2067608044213216 ) ) ;
#33796=PRODUCT_DEFINITION_SHAPE ( 'NONE', 'NONE',  #91591 ) ;
#33797=CARTESIAN_POINT ( 'NONE',  ( -3.133372182716995802, -284.3540076357942894, -336.0088801727681016 ) ) ;
#33798=CARTESIAN_POINT ( 'NONE',  ( -71.62570266975140498, -290.9214989012764931, -338.6488435612252488 ) ) ;
#33799=CARTESIAN_POINT ( 'NONE',  ( -45.95351796857004700, -290.4742168356576713, -346.4345253226774730 ) ) ;
#33800=CARTESIAN_POINT ( 'NONE',  ( -78.15830154116531503, -287.5039227347750739, -207.3788564912533445 ) ) ;
#33801=CARTESIAN_POINT ( 'NONE',  ( -25.39768465061203528, -280.3670567146467079, -194.2931188057497991 ) ) ;
#33802=CARTESIAN_POINT ( 'NONE',  ( -106.4459739295153042, -295.0308322974671569, -239.6718511773943590 ) ) ;
#33803=CARTESIAN_POINT ( 'NONE',  ( -76.75971970600521388, -283.3974967842848400, -336.5683819617340191 ) ) ;
#33805=CARTESIAN_POINT ( 'NONE',  ( 29.14719111883521663, -277.8541568506474846, -303.4936299544430653 ) ) ;
#33806=CARTESIAN_POINT ( 'NONE',  ( -53.35057174420112602, -276.3376638359844719, -200.3683826091709648 ) ) ;
#33807=CARTESIAN_POINT ( 'NONE',  ( 20.93880890519416127, -274.4569667345166977, -319.1192586699451113 ) ) ;
#33809=CARTESIAN_POINT ( 'NONE',  ( 20.56854496768234242, -280.4331769290819807, -225.7942674910315191 ) ) ;
#33811=CARTESIAN_POINT ( 'NONE',  ( -96.73673250947265956, -279.1044642454227755, -318.7576695002701399 ) ) ;
#33812=CARTESIAN_POINT ( 'NONE',  ( -83.12590738706026627, -284.5014538099298989, -208.6780673984494854 ) ) ;
#33813=CARTESIAN_POINT ( 'NONE',  ( -28.00036783105862881, -293.9323577414428428, -196.8881875353038424 ) ) ;
#33814=CARTESIAN_POINT ( 'NONE',  ( 29.84739320970582099, -277.6229826417745699, -306.4179061020159338 ) ) ;
#33816=CARTESIAN_POINT ( 'NONE',  ( -85.51080777927758447, -274.7169116835381715, -210.9217763012428009 ) ) ;
#33818=CARTESIAN_POINT ( 'NONE',  ( 32.09752579143857787, -275.6842649635597695, -292.8820839521200696 ) ) ;
#33820=CARTESIAN_POINT ( 'NONE',  ( -78.94842737287626733, -297.6142186612916021, -332.6242456462766768 ) ) ;
#33821=CARTESIAN_POINT ( 'NONE',  ( -111.8163763972752065, -282.6527165834509674, -262.5335868042495804 ) ) ;
#33822=CARTESIAN_POINT ( 'NONE',  ( 30.88215281240306354, -292.7574512093871135, -234.5917578125729506 ) ) ;
#33823=CARTESIAN_POINT ( 'NONE',  ( 29.34171850520809244, -273.1270556240142469, -236.8175868777147173 ) ) ;
#33824=CARTESIAN_POINT ( 'NONE',  ( 37.88852784372399185, -289.3094845643806821, -282.8007369110895866 ) ) ;
#33826=CARTESIAN_POINT ( 'NONE',  ( -33.47845432455119408, -291.0222134339394415, -197.1413233305401320 ) ) ;
#33828=CARTESIAN_POINT ( 'NONE',  ( -39.17918921479973449, -290.6042829835803900, -193.9595055652978886 ) ) ;
#33829=CARTESIAN_POINT ( 'NONE',  ( -110.3888421438364418, -290.2439803127227833, -268.4569745040915336 ) ) ;
#33831=CARTESIAN_POINT ( 'NONE',  ( 18.11841531099407021, -287.9038540202856211, -217.3159879620078243 ) ) ;
#33832=CARTESIAN_POINT ( 'NONE',  ( -96.42530883021679244, -279.4857723892326931, -227.4517405743245604 ) ) ;
#33833=CARTESIAN_POINT ( 'NONE',  ( -74.46881810041973893, -294.4539975366014914, -337.5255108577839565 ) ) ;
#33834=CARTESIAN_POINT ( 'NONE',  ( -110.8310821718662140, -285.4903081944621022, -247.5406397032579662 ) ) ;
#33835=CARTESIAN_POINT ( 'NONE',  ( 30.11098635295186909, -287.4036630030869901, -233.1576786375955805 ) ) ;
#33836=CARTESIAN_POINT ( 'NONE',  ( 21.83156336641219397, -282.4840437742049630, -313.1681846620591045 ) ) ;
#33837=CARTESIAN_POINT ( 'NONE',  ( 180.0122957173031182, 254.2448111356339666, -166.7447581597871817 ) ) ;
#33838=CARTESIAN_POINT ( 'NONE',  ( -72.14048337055831439, -195.4227484145153824, -359.3792095499467791 ) ) ;
#33839=CARTESIAN_POINT ( 'NONE',  ( -77.70721554921161101, -207.5803895343633201, -353.5487745245097244 ) ) ;
#33840=CARTESIAN_POINT ( 'NONE',  ( 35.80455650795468614, -274.7296725181265060, -268.8688490505106188 ) ) ;
#33841=CARTESIAN_POINT ( 'NONE',  ( 27.03163580294197388, -274.9505304558853709, -305.5428311301544682 ) ) ;
#33842=CARTESIAN_POINT ( 'NONE',  ( -54.57528130596574556, -297.3440671449835691, -195.3775825708489435 ) ) ;
#33843=CARTESIAN_POINT ( 'NONE',  ( -81.64875865379578102, -219.6352840722641702, -349.5921457167885933 ) ) ;
#33844=CARTESIAN_POINT ( 'NONE',  ( 37.10807293655612682, -274.4594436001175950, -288.0393427025508686 ) ) ;
#33845=CARTESIAN_POINT ( 'NONE',  ( -77.12757094218183340, -275.2710118047654078, -207.9507142341998644 ) ) ;
#33847=CARTESIAN_POINT ( 'NONE',  ( -70.63785974892620345, -298.5649740426521248, -201.1933077759243531 ) ) ;
#33848=CARTESIAN_POINT ( 'NONE',  ( 8.023052373463098519, -288.9048169349887303, -327.6326438215676262 ) ) ;
#33849=CARTESIAN_POINT ( 'NONE',  ( -111.0575757302146229, -297.0819044642089466, -292.0899524289468445 ) ) ;
#33850=CARTESIAN_POINT ( 'NONE',  ( -37.61374168157973941, -298.5411755449079578, -193.4231371344880586 ) ) ;
#33851=CARTESIAN_POINT ( 'NONE',  ( -9.729445409839209802, -292.5897147347177452, -202.7309814949156817 ) ) ;
#33853=CARTESIAN_POINT ( 'NONE',  ( 22.39492144971670129, -278.1020784981679981, -316.6514331525444845 ) ) ;
#33855=CARTESIAN_POINT ( 'NONE',  ( -11.52409435987599196, -279.8871164546936825, -197.8277467623605048 ) ) ;
#33857=CARTESIAN_POINT ( 'NONE',  ( -69.34344469044526704, -278.4250853560899372, -336.2483377748475846 ) ) ;
#33858=CARTESIAN_POINT ( 'NONE',  ( 12.06299619457478123, -278.1361065815718234, -328.0945571029552070 ) ) ;
#33859=CARTESIAN_POINT ( 'NONE',  ( -48.28068231435913304, -275.2106661057962356, -344.9708581079594296 ) ) ;
#33860=CARTESIAN_POINT ( 'NONE',  ( -108.5782377095010958, -297.4197250956665926, -253.9523282039501453 ) ) ;
#33861=CARTESIAN_POINT ( 'NONE',  ( -108.8760524274291299, -294.9002027674437727, -287.6831073336275040 ) ) ;
#33862=CARTESIAN_POINT ( 'NONE',  ( 37.92315709790361211, -281.8439440636951190, -254.3379082531501183 ) ) ;
#33863=CARTESIAN_POINT ( 'NONE',  ( -108.2901696014262853, -278.9455652831478005, -253.1763955837307947 ) ) ;
#33864=TOROIDAL_SURFACE ( 'NONE', #35427, 5.654241149514405151, 0.5000000000000000000 ) ;
#33865=CARTESIAN_POINT ( 'NONE',  ( -17.86612635525965942, -287.4909276363273420, -344.3476052467601107 ) ) ;
#33866=CARTESIAN_POINT ( 'NONE',  ( -37.62689429295477339, -300.0487446805060472, -195.1949880053350057 ) ) ;
#33868=CARTESIAN_POINT ( 'NONE',  ( -45.39034395246071796, -288.3539005628863947, -343.0785234603453091 ) ) ;
#33869=CONICAL_SURFACE ( 'NONE', #53537, 1.898405138727909947, 0.09862129276975308001 ) ;
#33870=CARTESIAN_POINT ( 'NONE',  ( -75.00236733635060205, -277.7834008169206186, -206.5868505137839293 ) ) ;
#33871=CARTESIAN_POINT ( 'NONE',  ( -94.38587109222731897, -277.7797112846501477, -223.8709310826332342 ) ) ;
#33872=CARTESIAN_POINT ( 'NONE',  ( -7.947696855606018573, -280.7438624002766687, -338.7519563420138979 ) ) ;
#33873=CARTESIAN_POINT ( 'NONE',  ( -109.0890889154887446, -286.8359154820719255, -248.3409727001177885 ) ) ;
#33874=CARTESIAN_POINT ( 'NONE',  ( -83.70035267687553926, -280.6048669847451720, -213.3918459106722310 ) ) ;
#33876=CARTESIAN_POINT ( 'NONE',  ( -30.89523986952798751, -294.1336568520080732, -195.5872849274080068 ) ) ;
#33878=CARTESIAN_POINT ( 'NONE',  ( -64.75075767896055368, -275.6449333277507776, -341.2878047447979384 ) ) ;
#33879=CARTESIAN_POINT ( 'NONE',  ( 11.82238302878409009, -276.9992650508387442, -324.5295881254055530 ) ) ;
#33880=CARTESIAN_POINT ( 'NONE',  ( 20.54221720100352400, -282.8919155636764344, -222.4082187477000900 ) ) ;
#33881=CARTESIAN_POINT ( 'NONE',  ( -112.5755490930345957, -292.5685981335822703, -262.8057246419418789 ) ) ;
#33882=CARTESIAN_POINT ( 'NONE',  ( -42.34388622391904988, -293.1150494231443417, -345.2067988781342365 ) ) ;
#33884=CARTESIAN_POINT ( 'NONE',  ( -69.71547127027052682, -284.8338905530135321, -200.6610764017653707 ) ) ;
#33886=CARTESIAN_POINT ( 'NONE',  ( -67.24291316677461339, -272.3365010762616976, -203.2119416307060931 ) ) ;
#33887=CARTESIAN_POINT ( 'NONE',  ( 29.86671287470853642, -291.2715533670002515, -238.7136208295203801 ) ) ;
#33890=CARTESIAN_POINT ( 'NONE',  ( -56.00034568096261012, -290.2961104416397689, -196.3163807350143202 ) ) ;
#33891=CARTESIAN_POINT ( 'NONE',  ( -95.60101743429282806, -286.7838469390944169, -225.0383577617677417 ) ) ;
#33892=CARTESIAN_POINT ( 'NONE',  ( 1.029587048623485046, -284.7967053985813664, -204.7592553813738903 ) ) ;
#33893=CARTESIAN_POINT ( 'NONE',  ( -103.5348021783674142, -285.5442206411549364, -302.6315960910006311 ) ) ;
#33895=CARTESIAN_POINT ( 'NONE',  ( -44.04933666083234556, -286.7680101382247813, -197.5077766789300995 ) ) ;
#33896=CARTESIAN_POINT ( 'NONE',  ( -6.581915198994430227, -294.4339016418616097, -201.5558411673713124 ) ) ;
#33897=CARTESIAN_POINT ( 'NONE',  ( 37.94362464737805851, -273.7140342564095477, -276.7980481195375546 ) ) ;
#33898=CARTESIAN_POINT ( 'NONE',  ( 38.90264903534559693, -275.7527198823302115, -259.7524652803982690 ) ) ;
#33899=CARTESIAN_POINT ( 'NONE',  ( -72.73710301352454621, -289.6670365382692012, -203.5896292693017244 ) ) ;
#33900=CARTESIAN_POINT ( 'NONE',  ( -112.9961795060496001, -278.7322726721104686, -255.9588285635283000 ) ) ;
#33901=CARTESIAN_POINT ( 'NONE',  ( -41.09731186905212041, -297.0795161791457986, -344.9242347159923270 ) ) ;
#33904=CARTESIAN_POINT ( 'NONE',  ( -42.69343914706002607, -284.6680750775250885, -197.0503691397170201 ) ) ;
#33905=CARTESIAN_POINT ( 'NONE',  ( 15.82382390753229373, -278.8044777029996908, -217.3881010388162451 ) ) ;
#33907=CARTESIAN_POINT ( 'NONE',  ( -10.57254070365111431, -272.8748510113835550, -198.8477803118141765 ) ) ;
#33908=CARTESIAN_POINT ( 'NONE',  ( -78.69649164067767799, -276.9739068929330301, -330.7027239114034955 ) ) ;
#33909=CARTESIAN_POINT ( 'NONE',  ( 23.51640978366198453, -295.6461198629912133, -312.0075538529216601 ) ) ;
#33910=CARTESIAN_POINT ( 'NONE',  ( -7.643943147984653130, -279.3527226730674329, -199.6394757744152173 ) ) ;
#33911=CARTESIAN_POINT ( 'NONE',  ( -42.39403018035636705, -296.0586874008787390, -343.4219310725983405 ) ) ;
#33912=CARTESIAN_POINT ( 'NONE',  ( -4.697651776471670537, -295.9462863609767282, -339.5684473380565009 ) ) ;
#33913=CARTESIAN_POINT ( 'NONE',  ( -44.56697264216801813, -297.7916432804731812, -197.6691815334732212 ) ) ;
#33914=CARTESIAN_POINT ( 'NONE',  ( -52.80637680195250994, -293.8542785132333961, -196.9194786388742671 ) ) ;
#33915=CARTESIAN_POINT ( 'NONE',  ( -99.34550382253182477, -285.3263917739964199, -224.6167497834574931 ) ) ;
#33916=CARTESIAN_POINT ( 'NONE',  ( 36.09394618947436584, -273.4546752615383411, -251.7194621177667386 ) ) ;
#33917=CARTESIAN_POINT ( 'NONE',  ( -37.50372076829603429, -288.8874127097809037, -347.3740193428915290 ) ) ;
#33918=CARTESIAN_POINT ( 'NONE',  ( -112.0377693549130385, -280.5280725484354321, -270.6694575696985794 ) ) ;
#33919=CARTESIAN_POINT ( 'NONE',  ( 32.53451506376017477, -286.9025561681858107, -292.4552068991233114 ) ) ;
#33920=CARTESIAN_POINT ( 'NONE',  ( -40.52145238496140678, -290.0120326608300161, -195.4157094716535710 ) ) ;
#33921=CARTESIAN_POINT ( 'NONE',  ( -72.76141013609318975, -193.8959084914727669, -354.0272458012134393 ) ) ;
#33923=CARTESIAN_POINT ( 'NONE',  ( 17.82677097956141310, -286.3775288375660466, -222.4609276129978070 ) ) ;
#33925=CARTESIAN_POINT ( 'NONE',  ( 36.96706595943278018, -282.7352201434646304, -289.6231920196497072 ) ) ;
#33926=CARTESIAN_POINT ( 'NONE',  ( -114.1548182960137154, -289.6002006125409025, -271.2141424905611302 ) ) ;
#33927=CARTESIAN_POINT ( 'NONE',  ( 34.56590657953351098, -282.8291154953886348, -244.9898298213585122 ) ) ;
#33928=EDGE_CURVE ( 'NONE', #47026, #65957, #21855, .T. ) ;
#33929=CARTESIAN_POINT ( 'NONE',  ( -5.166719963894286671, -281.7820234821972463, -200.9488069267982269 ) ) ;
#33930=CARTESIAN_POINT ( 'NONE',  ( 33.32297546006198274, -281.6278747319022386, -288.7276615407365625 ) ) ;
#33931=CARTESIAN_POINT ( 'NONE',  ( 4.012042091634596019, -276.6089133121712962, -207.7301516251787632 ) ) ;
#33932=CARTESIAN_POINT ( 'NONE',  ( -58.85132075442897559, -295.3227910122868138, -344.3513654065019978 ) ) ;
#33934=CARTESIAN_POINT ( 'NONE',  ( -99.65911228022191892, -289.1307003409116874, -229.1772899730015638 ) ) ;
#33935=CARTESIAN_POINT ( 'NONE',  ( -49.99381059216882051, -296.8072274659227219, -198.1520453282938377 ) ) ;
#33937=ORIENTED_EDGE ( 'NONE', *, *, #70497, .T. ) ;
#33938=CARTESIAN_POINT ( 'NONE',  ( -104.8005769654177470, -286.8905090258740529, -238.7648156088026496 ) ) ;
#33940=CARTESIAN_POINT ( 'NONE',  ( -6.025790800353265197, -293.5338264351685780, -200.3411290667411890 ) ) ;
#33942=CARTESIAN_POINT ( 'NONE',  ( 21.09638085842285449, -282.8196341261192970, -314.3008608180597321 ) ) ;
#33943=CARTESIAN_POINT ( 'NONE',  ( 22.58222267754217683, -273.9660599147180164, -222.3616934020354563 ) ) ;
#33944=CARTESIAN_POINT ( 'NONE',  ( -56.17186648268803850, -292.4672961695368372, -195.7492988734259143 ) ) ;
#33945=CARTESIAN_POINT ( 'NONE',  ( -112.6782060976187125, -282.5894872960722068, -278.4057651175401702 ) ) ;
#33946=CARTESIAN_POINT ( 'NONE',  ( -36.38289612213738877, -292.3971445684914556, -193.3752045111904465 ) ) ;
#33947=CARTESIAN_POINT ( 'NONE',  ( 35.67636106844881994, -287.8942844350714836, -271.0321066393260594 ) ) ;
#33951=CARTESIAN_POINT ( 'NONE',  ( -30.58931055946544930, -124.9542506483939661, -360.4434141177968058 ) ) ;
#33952=CARTESIAN_POINT ( 'NONE',  ( -68.88204076869831738, -284.9794498174313730, -339.8585973204147876 ) ) ;
#33953=CARTESIAN_POINT ( 'NONE',  ( -37.37352853689063181, -286.5523547857347353, -345.3611179825600175 ) ) ;
#33955=CARTESIAN_POINT ( 'NONE',  ( 33.75873697741572244, -280.2371728747124280, -252.4507961944683530 ) ) ;
#33956=CARTESIAN_POINT ( 'NONE',  ( -17.36747659711747716, -276.4679232909452935, -344.7033985890554391 ) ) ;
#33957=CARTESIAN_POINT ( 'NONE',  ( -110.9396822562341072, -280.7265676173724955, -256.8198678388772578 ) ) ;
#33958=CARTESIAN_POINT ( 'NONE',  ( -28.99645464915736426, -125.7048492729908844, -362.1742968396590641 ) ) ;
#33959=CARTESIAN_POINT ( 'NONE',  ( 38.93968215176566616, -280.1933904221051534, -275.6384269944435914 ) ) ;
#33960=CARTESIAN_POINT ( 'NONE',  ( -111.8687854989046713, -282.6371639646095559, -265.3297698834770699 ) ) ;
#33961=CARTESIAN_POINT ( 'NONE',  ( 74.50552286126109891, -301.1943555422959093, -194.3414303693253942 ) ) ;
#33962=CARTESIAN_POINT ( 'NONE',  ( 27.21538126783730505, -294.5114283558988859, -304.6799393237983509 ) ) ;
#33964=CARTESIAN_POINT ( 'NONE',  ( -88.26027104274552926, -290.0060137901919575, -217.2951193044740421 ) ) ;
#33965=CARTESIAN_POINT ( 'NONE',  ( 36.39808021849354702, -276.4780918186856411, -292.2194611461752629 ) ) ;
#33966=CARTESIAN_POINT ( 'NONE',  ( 34.62565556512682008, -275.3897703403181367, -258.0516880542799640 ) ) ;
#33967=CARTESIAN_POINT ( 'NONE',  ( -105.3285225304123429, -271.9334142874049007, -234.7599817635760076 ) ) ;
#33971=CARTESIAN_POINT ( 'NONE',  ( -32.10997743103977342, -284.0642804638028451, -343.4833112722011492 ) ) ;
#33972=CARTESIAN_POINT ( 'NONE',  ( 28.39852645911823359, -282.8100872159531605, -232.2534203327600153 ) ) ;
#33973=CARTESIAN_POINT ( 'NONE',  ( -107.4920760518732124, -283.6285397354857309, -290.9683537902830039 ) ) ;
#33974=CARTESIAN_POINT ( 'NONE',  ( 16.03938483626188116, -273.2242654959118227, -219.3273305455436741 ) ) ;
#33975=CARTESIAN_POINT ( 'NONE',  ( 34.29949583178225225, -283.1593043212120051, -250.8599200980146122 ) ) ;
#33976=CARTESIAN_POINT ( 'NONE',  ( 25.88051309963617186, -273.5149583736509840, -232.3985397861895024 ) ) ;
#33979=CARTESIAN_POINT ( 'NONE',  ( 33.19903817164158966, -276.8950740075472368, -290.3627966629713342 ) ) ;
#33981=CARTESIAN_POINT ( 'NONE',  ( -7.936953301847952780, -277.4794296980350623, -341.3649480753508669 ) ) ;
#33984=CARTESIAN_POINT ( 'NONE',  ( -112.9215738670834810, -286.4887184956436386, -264.3698898999080029 ) ) ;
#33985=CARTESIAN_POINT ( 'NONE',  ( -53.19430546647188152, -294.4576817735630812, -341.8365809690592414 ) ) ;
#33986=CARTESIAN_POINT ( 'NONE',  ( -40.34309663412894054, -288.4375128050641024, -347.2136539543908498 ) ) ;
#33987=CARTESIAN_POINT ( 'NONE',  ( -54.97635030180521909, -284.0622926803411019, -198.4262982381889913 ) ) ;
#33988=CARTESIAN_POINT ( 'NONE',  ( -88.08780951512318325, -283.8996518100920525, -217.0675226988815893 ) ) ;
#33989=CARTESIAN_POINT ( 'NONE',  ( -66.75203379905119050, -287.6825588362717099, -338.3350088139837339 ) ) ;
#33990=CARTESIAN_POINT ( 'NONE',  ( -73.98177366119345777, -284.7552141577755833, -334.0164782382196904 ) ) ;
#33991=CARTESIAN_POINT ( 'NONE',  ( 19.29282285170698685, -274.2343777784859640, -319.5489460889735938 ) ) ;
#33992=CARTESIAN_POINT ( 'NONE',  ( 2.341958187015649173, -284.9744114329763534, -205.3100020999200126 ) ) ;
#33993=CARTESIAN_POINT ( 'NONE',  ( -109.6994976599125238, -298.8082655502121838, -250.4370192811250035 ) ) ;
#33994=CARTESIAN_POINT ( 'NONE',  ( 21.57126856253321279, -284.9118906762126358, -223.6577211002585557 ) ) ;
#33995=CARTESIAN_POINT ( 'NONE',  ( -22.15728714507084263, -281.1925723890024642, -198.6652394722845543 ) ) ;
#33996=CARTESIAN_POINT ( 'NONE',  ( 13.38570060246112625, -290.3449888207655931, -325.9002156649412996 ) ) ;
#33999=CARTESIAN_POINT ( 'NONE',  ( -95.38917135227156052, -297.8090270661739964, -318.7527617647824059 ) ) ;
#34000=CARTESIAN_POINT ( 'NONE',  ( -107.3728874697466864, -276.9026434713559865, -243.3711692907941710 ) ) ;
#34001=CARTESIAN_POINT ( 'NONE',  ( -39.19752279556439589, -291.2266220305182287, -193.5320000469215529 ) ) ;
#34002=CARTESIAN_POINT ( 'NONE',  ( -100.8653498173375311, -294.4402680124741210, -308.0275480268938963 ) ) ;
#34003=CARTESIAN_POINT ( 'NONE',  ( -36.98926432934193542, -278.7414808409349689, -196.8688104348144066 ) ) ;
#34004=CARTESIAN_POINT ( 'NONE',  ( -24.32098240830451275, -272.2993628225917178, -197.0161142878270937 ) ) ;
#34005=CARTESIAN_POINT ( 'NONE',  ( 35.69898607080695285, -294.9798952575358157, -278.9516643286306135 ) ) ;
#34006=CARTESIAN_POINT ( 'NONE',  ( -37.30987171927208124, -291.5519495502701943, -345.3611179825600175 ) ) ;
#34007=CARTESIAN_POINT ( 'NONE',  ( -113.0842082891596192, -295.1489164937283363, -261.0993573750959627 ) ) ;
#34008=CARTESIAN_POINT ( 'NONE',  ( -70.43586177752509059, -289.8617341429207954, -201.9597255801413382 ) ) ;
#34011=CARTESIAN_POINT ( 'NONE',  ( -100.2244542782971877, -292.4996399343670532, -232.1363335249015734 ) ) ;
#34013=CARTESIAN_POINT ( 'NONE',  ( -102.5581352461478417, -291.8056555447890901, -237.0914645410217361 ) ) ;
#34015=CARTESIAN_POINT ( 'NONE',  ( -79.38935137501394479, -292.7034758802020633, -206.2664310017685807 ) ) ;
#34016=CARTESIAN_POINT ( 'NONE',  ( 22.92416737053131826, -280.1875310139956810, -315.5986247710465022 ) ) ;
#34017=CARTESIAN_POINT ( 'NONE',  ( 34.90773852373655473, -293.4144154234762709, -259.9199200389712701 ) ) ;
#34018=CARTESIAN_POINT ( 'NONE',  ( 34.32442234620443600, -281.1935247373220363, -242.0559225940189947 ) ) ;
#34019=CARTESIAN_POINT ( 'NONE',  ( -79.15180197502634485, -283.2665206669882991, -334.9959358056071324 ) ) ;
#34020=CARTESIAN_POINT ( 'NONE',  ( -2.535806182505966788, -286.5909035716658764, -336.6648404453312651 ) ) ;
#34021=CARTESIAN_POINT ( 'NONE',  ( -68.32107128253467465, -281.6030802125077344, -337.8232854999885149 ) ) ;
#34022=CARTESIAN_POINT ( 'NONE',  ( -40.95601238282657874, -278.4873620651294459, -194.1270171780464864 ) ) ;
#34024=CARTESIAN_POINT ( 'NONE',  ( -15.48832416722109784, -285.2487406300211887, -196.7945681685554291 ) ) ;
#34026=CARTESIAN_POINT ( 'NONE',  ( 30.58417658934985894, -294.7675374175377669, -241.3771148903026642 ) ) ;
#34027=CARTESIAN_POINT ( 'NONE',  ( 38.96474186452985577, -276.9156468500540882, -265.4593488087880928 ) ) ;
#34028=CARTESIAN_POINT ( 'NONE',  ( -59.20537098553337074, -277.0098052680232286, -340.0322553591669816 ) ) ;
#34029=CARTESIAN_POINT ( 'NONE',  ( -114.2511981872462172, -290.6721558643066032, -274.0932906438868031 ) ) ;
#34030=CARTESIAN_POINT ( 'NONE',  ( -69.87274048461915754, -281.5569754628715486, -338.5738857300366931 ) ) ;
#34032=CARTESIAN_POINT ( 'NONE',  ( 35.06877942850390895, -292.7593506057716013, -281.6510474007383209 ) ) ;
#34033=CARTESIAN_POINT ( 'NONE',  ( -108.4575962103301521, -294.2440151453465091, -294.1840055613633353 ) ) ;
#34036=CARTESIAN_POINT ( 'NONE',  ( 20.23526115831166905, -292.4261569162461001, -225.3644017674343161 ) ) ;
#34038=CARTESIAN_POINT ( 'NONE',  ( 34.45848030099739390, -285.0523547857347353, -270.3937649182068412 ) ) ;
#34039=CARTESIAN_POINT ( 'NONE',  ( -103.6405245513603006, -296.1171399088249814, -231.5616079269409795 ) ) ;
#34040=CARTESIAN_POINT ( 'NONE',  ( -4.176559497390433862, -278.6242926352928180, -202.2265031768656911 ) ) ;
#34041=CARTESIAN_POINT ( 'NONE',  ( -54.86800706650167569, -287.1465538443983974, -195.8887953618685458 ) ) ;
#34042=CARTESIAN_POINT ( 'NONE',  ( -22.45776154617337284, -286.0812411442398115, -198.8426827372608727 ) ) ;
#34043=CARTESIAN_POINT ( 'NONE',  ( -85.54426511926337184, -279.2528950300395536, -326.1711458074203733 ) ) ;
#34044=CARTESIAN_POINT ( 'NONE',  ( -71.71005442459195933, -293.5286674088560517, -336.6374977733872811 ) ) ;
#34045=CARTESIAN_POINT ( 'NONE',  ( -110.7441574846909589, -298.4408178982099571, -260.4834188170263474 ) ) ;
#34046=CARTESIAN_POINT ( 'NONE',  ( -68.21835684903309982, -276.2618711082805589, -336.9614464224553672 ) ) ;
#34049=CARTESIAN_POINT ( 'NONE',  ( -114.0993797465282000, -296.3000993316945824, -263.8680149877381496 ) ) ;
#34050=CARTESIAN_POINT ( 'NONE',  ( -56.41134552392333035, -291.2198180045460276, -342.3706854506460218 ) ) ;
#34051=CARTESIAN_POINT ( 'NONE',  ( -113.9811632769476972, -273.7037598431215883, -270.3757807067846670 ) ) ;
#34053=CARTESIAN_POINT ( 'NONE',  ( -42.66306414405371328, -289.7723305437850740, -343.3197876190436091 ) ) ;
#34056=CARTESIAN_POINT ( 'NONE',  ( 39.29344655529643404, -280.6773327982243700, -275.6566465591066617 ) ) ;
#34057=CARTESIAN_POINT ( 'NONE',  ( -97.27212975846579468, -297.8501493462121630, -222.1775482569719600 ) ) ;
#34058=CARTESIAN_POINT ( 'NONE',  ( -67.80994736009630230, -289.7961396489703247, -200.9784651223534695 ) ) ;
#34059=CARTESIAN_POINT ( 'NONE',  ( -91.62362531028934143, -297.6373943008153446, -215.7789149307212426 ) ) ;
#34060=CARTESIAN_POINT ( 'NONE',  ( 22.95284970476897612, -294.4594706035056788, -311.6400159918918575 ) ) ;
#34064=CARTESIAN_POINT ( 'NONE',  ( -40.29239099905376520, -290.6086970247865793, -346.6236799829580377 ) ) ;
#34065=CARTESIAN_POINT ( 'NONE',  ( -115.3430155898818299, -275.2662352645559167, -252.5904736702033517 ) ) ;
#34066=CARTESIAN_POINT ( 'NONE',  ( 24.16857221796717070, -281.5157951686662159, -316.5108653582693705 ) ) ;
#34067=CARTESIAN_POINT ( 'NONE',  ( -74.48724569931793837, -287.5570800579903903, -205.3829050902639892 ) ) ;
#34068=CARTESIAN_POINT ( 'NONE',  ( -30.91518192134769194, -284.7065671193287244, -194.2078817765512326 ) ) ;
#34069=CARTESIAN_POINT ( 'NONE',  ( -82.14886478029592354, -271.4397368046327301, -210.3599260659470076 ) ) ;
#34070=CARTESIAN_POINT ( 'NONE',  ( -57.27018824581460166, -275.7133050650101609, -198.5844903303144235 ) ) ;
#34071=CARTESIAN_POINT ( 'NONE',  ( -109.1343325549277949, -288.8869285131793845, -250.6854444463411085 ) ) ;
#34072=CARTESIAN_POINT ( 'NONE',  ( -105.2279313368564857, -279.9717745156498268, -304.1207988128684860 ) ) ;
#34075=CARTESIAN_POINT ( 'NONE',  ( -74.50578879177095359, -279.5432581245993333, -207.4712528357910628 ) ) ;
#34076=CARTESIAN_POINT ( 'NONE',  ( 0.4597544453736828185, -279.9185308260847478, -207.7330151771021463 ) ) ;
#34077=CARTESIAN_POINT ( 'NONE',  ( -41.35446724305695199, -278.1812004345095488, -346.9601094228135025 ) ) ;
#34078=CARTESIAN_POINT ( 'NONE',  ( -98.25125140309884841, -277.9698254411319454, -223.8850971725964598 ) ) ;
#34079=CARTESIAN_POINT ( 'NONE',  ( 23.96410439411992144, -22.95231442736623961, -342.3546796976241922 ) ) ;
#34080=CARTESIAN_POINT ( 'NONE',  ( -31.29060213888120501, -275.0680370213951846, -193.8220356742286867 ) ) ;
#34081=CARTESIAN_POINT ( 'NONE',  ( -113.6490859602314458, -274.1078910969521871, -267.5387840032006466 ) ) ;
#34082=CARTESIAN_POINT ( 'NONE',  ( -95.99890600148557951, -287.6948066931273615, -223.6242672951989618 ) ) ;
#34085=CARTESIAN_POINT ( 'NONE',  ( 33.38377129521822440, -288.8878382860228839, -289.8403967537881840 ) ) ;
#34086=CARTESIAN_POINT ( 'NONE',  ( 37.67825218094539252, -289.4694715674509666, -282.7638406731388159 ) ) ;
#34087=CARTESIAN_POINT ( 'NONE',  ( -107.8480086104094511, -290.1554643315773774, -251.0543022790026555 ) ) ;
#34089=CARTESIAN_POINT ( 'NONE',  ( -94.35776859030636388, -283.3573122073266290, -322.0400717641096549 ) ) ;
#34090=CARTESIAN_POINT ( 'NONE',  ( -24.71974998225321585, -278.6157439033871697, -197.6484864261477128 ) ) ;
#34091=CARTESIAN_POINT ( 'NONE',  ( -6.525001032820303415, -288.3216011438467490, -202.8105302942128674 ) ) ;
#34092=CARTESIAN_POINT ( 'NONE',  ( 21.55244503841817760, -280.6484501256633735, -314.6785487041663032 ) ) ;
#34093=CARTESIAN_POINT ( 'NONE',  ( -62.49335387163878863, -281.0332462661451132, -201.2520706272952680 ) ) ;
#34094=CARTESIAN_POINT ( 'NONE',  ( -94.49725744858243104, -278.4021019860585966, -315.8918755371297493 ) ) ;
#34095=CARTESIAN_POINT ( 'NONE',  ( -110.0491350529586896, -289.6541086403312875, -246.0780596479599467 ) ) ;
#34097=CARTESIAN_POINT ( 'NONE',  ( -97.91081248409466298, -284.7218857487312107, -317.6426307511187019 ) ) ;
#34098=CARTESIAN_POINT ( 'NONE',  ( -70.43795861538282566, -283.9690859577434594, -339.8317737581044184 ) ) ;
#34099=CARTESIAN_POINT ( 'NONE',  ( 32.73399436149124853, -281.4482396454762920, -249.9063619019148064 ) ) ;
#34102=CARTESIAN_POINT ( 'NONE',  ( -112.5839257842204120, -292.2941684954919879, -279.6763025183694822 ) ) ;
#34103=CARTESIAN_POINT ( 'NONE',  ( -53.27018935036315384, -290.5369703425506600, -195.4766199927961736 ) ) ;
#34104=CARTESIAN_POINT ( 'NONE',  ( -5.193986013452473571, -273.5447278070696484, -204.5450220920763513 ) ) ;
#34105=CARTESIAN_POINT ( 'NONE',  ( -92.62948948336432409, -295.1676020695161924, -323.8080368340068276 ) ) ;
#34106=CARTESIAN_POINT ( 'NONE',  ( -105.3353714735707456, -289.4112212900803911, -241.8106601527474879 ) ) ;
#34107=CARTESIAN_POINT ( 'NONE',  ( -92.96686275007328959, -294.1046335545701140, -319.1854489888458488 ) ) ;
#34108=CARTESIAN_POINT ( 'NONE',  ( -50.80934700523397396, -290.4329906233576253, -342.5639802035804564 ) ) ;
#34110=CARTESIAN_POINT ( 'NONE',  ( -112.0180864730158135, -292.6485916659394775, -262.8629131661964493 ) ) ;
#34111=CARTESIAN_POINT ( 'NONE',  ( 34.94817831876405023, -291.2869794180836607, -249.7179989626914676 ) ) ;
#34112=CARTESIAN_POINT ( 'NONE',  ( 0.1456907602883386610, -296.5536393596636344, -335.3792260792246225 ) ) ;
#34113=CARTESIAN_POINT ( 'NONE',  ( -41.34774620322242811, -286.9417676393394459, -197.2229338460356587 ) ) ;
#34114=CARTESIAN_POINT ( 'NONE',  ( 18.19280791292056065, -296.2584298847453965, -321.0921382488502900 ) ) ;
#34115=CARTESIAN_POINT ( 'NONE',  ( -10.94785911146214907, -276.3743007225289716, -199.7239453671863316 ) ) ;
#34116=CARTESIAN_POINT ( 'NONE',  ( -101.4093944506181231, -296.3087734224329779, -227.9167751567856612 ) ) ;
#34117=CARTESIAN_POINT ( 'NONE',  ( 34.21625681899154614, -274.0382403512223277, -289.2670115886104441 ) ) ;
#34118=CARTESIAN_POINT ( 'NONE',  ( -27.34117906137161924, -278.2599127589096497, -196.5437218858108110 ) ) ;
#34119=CARTESIAN_POINT ( 'NONE',  ( -63.46229987583587473, -274.9091260301817101, -201.7556787663423847 ) ) ;
#34120=CARTESIAN_POINT ( 'NONE',  ( -73.57685916769965218, -296.9684271807299751, -334.4110060935207116 ) ) ;
#34122=CARTESIAN_POINT ( 'NONE',  ( -109.8977365114597831, -297.4836636431418242, -260.5852763454557248 ) ) ;
#34124=CARTESIAN_POINT ( 'NONE',  ( 6.946997655045254128, -286.4731799766560130, -331.3919821122094618 ) ) ;
#34125=CARTESIAN_POINT ( 'NONE',  ( -39.16832825069231205, -298.0286293834245157, -197.3715658859814255 ) ) ;
#34126=CARTESIAN_POINT ( 'NONE',  ( -18.18202730792959798, -286.2923489644513779, -195.7278220891037108 ) ) ;
#34127=CARTESIAN_POINT ( 'NONE',  ( -106.4963837127592114, -289.7831786279602966, -304.2961098652312444 ) ) ;
#34128=CARTESIAN_POINT ( 'NONE',  ( -101.6974943702453231, -298.0089557341152613, -309.5623749605413195 ) ) ;
#34129=CARTESIAN_POINT ( 'NONE',  ( 18.43033625258885877, -292.2484930883596235, -320.2754033582658622 ) ) ;
#34130=CARTESIAN_POINT ( 'NONE',  ( 10.72996806318832697, -279.8942709253076373, -210.3489928628017083 ) ) ;
#34131=CARTESIAN_POINT ( 'NONE',  ( 35.77081079830085031, -291.2666405000204577, -287.0812184334320705 ) ) ;
#34132=CARTESIAN_POINT ( 'NONE',  ( -31.99008365135278709, -278.1193823247964474, -195.5011384472874738 ) ) ;
#34134=CARTESIAN_POINT ( 'NONE',  ( -26.43093704204658678, -287.7052756228085855, -342.9940240511675142 ) ) ;
#34136=CARTESIAN_POINT ( 'NONE',  ( -59.29832019713345659, -287.3360734160912671, -342.1294428259476490 ) ) ;
#34137=CARTESIAN_POINT ( 'NONE',  ( -95.08992131036499984, -298.7941371276687619, -224.4091499278419519 ) ) ;
#34138=CARTESIAN_POINT ( 'NONE',  ( 26.24172034550992905, -283.5394810421779539, -312.7374667348826165 ) ) ;
#34139=CARTESIAN_POINT ( 'NONE',  ( -23.70543015075491766, -296.2421586485600074, -195.0104836624347229 ) ) ;
#34140=CARTESIAN_POINT ( 'NONE',  ( -7.253477599204388504, -282.6461819827468958, -336.8857243858190031 ) ) ;
#34141=CARTESIAN_POINT ( 'NONE',  ( -100.0072663391817116, -296.1251220170856300, -315.1949358746243206 ) ) ;
#34142=CARTESIAN_POINT ( 'NONE',  ( -85.71101201707695338, -274.7927557365734970, -214.8334300653035029 ) ) ;
#34143=CARTESIAN_POINT ( 'NONE',  ( -38.17394810588402265, -282.0418783422173874, -195.3657313487321971 ) ) ;
#34145=CARTESIAN_POINT ( 'NONE',  ( -65.92102631255339418, -272.5895162221976875, -202.8522430917905979 ) ) ;
#34148=CARTESIAN_POINT ( 'NONE',  ( -103.7121307357248270, -286.9861502599965775, -236.2024771924168647 ) ) ;
#34150=CARTESIAN_POINT ( 'NONE',  ( -88.47809603358389552, -270.9094976428775681, -206.1857440867352693 ) ) ;
#34151=CARTESIAN_POINT ( 'NONE',  ( 39.54570447168232050, -274.7595855121853674, -271.1801476732283049 ) ) ;
#34152=CARTESIAN_POINT ( 'NONE',  ( -95.79067256070787550, -288.2870132970578538, -319.2706062192905279 ) ) ;
#34153=CARTESIAN_POINT ( 'NONE',  ( -89.37021202850928603, -285.3208969136950373, -322.6222017936670454 ) ) ;
#34155=CARTESIAN_POINT ( 'NONE',  ( 22.92245501723914103, -276.5638357021172737, -227.7402827711986220 ) ) ;
#34156=CARTESIAN_POINT ( 'NONE',  ( -68.92619799722855589, -284.8846154903290540, -339.9529003934567868 ) ) ;
#34157=CARTESIAN_POINT ( 'NONE',  ( -70.40747916372360748, -282.2929650765553902, -335.9021511718655688 ) ) ;
#34158=CARTESIAN_POINT ( 'NONE',  ( -63.01692027197296397, -281.7181222955002227, -199.8379734364742149 ) ) ;
#34159=CARTESIAN_POINT ( 'NONE',  ( 22.75701880966415303, -275.0738125612895146, -222.2034882017491668 ) ) ;
#34160=CARTESIAN_POINT ( 'NONE',  ( 19.87577994980237150, -276.0851004532101456, -321.9090938423320267 ) ) ;
#34161=CARTESIAN_POINT ( 'NONE',  ( -72.78917252419117290, -297.4455974563690575, -335.8339804502215884 ) ) ;
#34162=CARTESIAN_POINT ( 'NONE',  ( 202.9738562182569694, 291.4636489450776367, -54.00000000000002132 ) ) ;
#34165=CARTESIAN_POINT ( 'NONE',  ( -97.31153091690073609, -294.0636545742849535, -316.6636544058733307 ) ) ;
#34166=CARTESIAN_POINT ( 'NONE',  ( 35.64881279390860414, -275.0041870897437661, -266.1416613042164840 ) ) ;
#34167=CARTESIAN_POINT ( 'NONE',  ( -112.0594013691240320, -273.9695499620431178, -253.4710664164755940 ) ) ;
#34168=CARTESIAN_POINT ( 'NONE',  ( -72.88000030762979975, -287.3347175841545322, -205.4236458839362740 ) ) ;
#34169=CARTESIAN_POINT ( 'NONE',  ( 0.2162673356445698469, -296.0816087897763396, -336.7998545558571095 ) ) ;
#34170=CARTESIAN_POINT ( 'NONE',  ( -22.16114993015452939, -296.0669233517037355, -345.4448020502308054 ) ) ;
#34171=CARTESIAN_POINT ( 'NONE',  ( -107.7490710117445047, -292.2229007735709843, -295.7152212084682787 ) ) ;
#34172=CARTESIAN_POINT ( 'NONE',  ( -32.82759728356906948, -278.1090144360034060, -195.6640544304578384 ) ) ;
#34173=CARTESIAN_POINT ( 'NONE',  ( -92.37762154732315878, -281.1770942952284713, -220.2376548908851532 ) ) ;
#34174=CARTESIAN_POINT ( 'NONE',  ( -69.15452005819952319, -293.5536797952444203, -337.6748891966883548 ) ) ;
#34175=CARTESIAN_POINT ( 'NONE',  ( -105.8780573088721439, -285.9921136731020965, -302.6577621141794339 ) ) ;
#34176=CARTESIAN_POINT ( 'NONE',  ( -96.81759069273830676, -284.0695546312793454, -227.4812839670699418 ) ) ;
#34177=CARTESIAN_POINT ( 'NONE',  ( 203.7321165250324668, 291.7437209203117732, -83.00941222436438238 ) ) ;
#34179=CARTESIAN_POINT ( 'NONE',  ( -110.4116108969717800, -284.2116931893817764, -270.9052225107727736 ) ) ;
#34181=CARTESIAN_POINT ( 'NONE',  ( 23.49367090263939062, -282.0061579582571767, -223.6433084205988848 ) ) ;
#34182=CARTESIAN_POINT ( 'NONE',  ( -100.7382298977241675, -273.3829978328583366, -234.0245348386029320 ) ) ;
#34183=CARTESIAN_POINT ( 'NONE',  ( 32.35715484267636555, -285.9372595385578393, -238.4516400640781342 ) ) ;
#34184=CARTESIAN_POINT ( 'NONE',  ( 24.39535264029694872, -281.8852234763402862, -224.7392314696223252 ) ) ;
#34185=CARTESIAN_POINT ( 'NONE',  ( -28.66051455370715217, -278.4642198410956553, -346.2254563204683109 ) ) ;
#34186=CARTESIAN_POINT ( 'NONE',  ( -7.584104958080704506, -281.0835276684457540, -199.4398651030447809 ) ) ;
#34187=CARTESIAN_POINT ( 'NONE',  ( -82.13390479932374433, -275.1952119285919025, -326.4764044574609443 ) ) ;
#34188=CARTESIAN_POINT ( 'NONE',  ( 186.3365424865488649, 263.1243791769486506, -153.3719034750679668 ) ) ;
#34190=CARTESIAN_POINT ( 'NONE',  ( -8.281836757531388926, -276.4335520200463634, -201.3453464442936536 ) ) ;
#34191=CARTESIAN_POINT ( 'NONE',  ( -96.00831230668778460, -239.6785672792925084, -341.5384560403468299 ) ) ;
#34192=CARTESIAN_POINT ( 'NONE',  ( -96.06964175806390926, -277.2078255921074970, -224.2658797213836408 ) ) ;
#34193=CARTESIAN_POINT ( 'NONE',  ( 37.08269106238812185, -295.5065568923598676, -285.6903062367455277 ) ) ;
#34194=CARTESIAN_POINT ( 'NONE',  ( -96.49577611763895391, -295.3002576149756351, -313.3323175975022536 ) ) ;
#34195=CARTESIAN_POINT ( 'NONE',  ( -19.39503787202268725, -291.7845599245733865, -195.4902691391098983 ) ) ;
#34197=CARTESIAN_POINT ( 'NONE',  ( -69.29815934365844043, -294.0391298202816870, -339.7828701516911565 ) ) ;
#34198=CARTESIAN_POINT ( 'NONE',  ( 36.48117793508753692, -285.9252560597526553, -268.3103397172464497 ) ) ;
#34199=CARTESIAN_POINT ( 'NONE',  ( 0.5189787395971917627, -294.4229559535997964, -206.5063258683094887 ) ) ;
#34200=CARTESIAN_POINT ( 'NONE',  ( -100.8187061040173518, -285.3623745025093399, -307.4004644863990166 ) ) ;
#34202=CARTESIAN_POINT ( 'NONE',  ( -22.25180916154481636, -293.1819847042034439, -195.0399983904050885 ) ) ;
#34203=CARTESIAN_POINT ( 'NONE',  ( -10.94769166799071236, -283.1910222452466428, -338.5421615008685876 ) ) ;
#34204=CARTESIAN_POINT ( 'NONE',  ( -108.0146749630194876, -294.9677151944059688, -300.0507857283180329 ) ) ;
#34205=CARTESIAN_POINT ( 'NONE',  ( -101.5546552396239832, -291.9119650482858788, -228.0654395753772405 ) ) ;
#34206=CARTESIAN_POINT ( 'NONE',  ( -54.48180009559617076, -289.7588846097125952, -345.4207441679834574 ) ) ;
#34207=CARTESIAN_POINT ( 'NONE',  ( 0.1668406292046996364, -286.7329591081249873, -207.6754406805349618 ) ) ;
#34210=CARTESIAN_POINT ( 'NONE',  ( -104.8462350135037298, -297.9610003366339015, -304.8778264340903661 ) ) ;
#34211=CARTESIAN_POINT ( 'NONE',  ( -107.3151688544295439, -295.6357149952872874, -239.2945897424149280 ) ) ;
#34212=CARTESIAN_POINT ( 'NONE',  ( -14.22327118428249193, -279.4180640100485675, -200.8168802035525289 ) ) ;
#34213=CARTESIAN_POINT ( 'NONE',  ( 37.17757660505726847, -275.2995487761617710, -289.5028080494026881 ) ) ;
#34214=CARTESIAN_POINT ( 'NONE',  ( -63.30579144633913558, -296.1876606117900224, -201.3392190997583953 ) ) ;
#34215=CARTESIAN_POINT ( 'NONE',  ( 6.139126437467123054, -278.3158928617020820, -330.5933993505445869 ) ) ;
#34216=CARTESIAN_POINT ( 'NONE',  ( 36.58190275923615786, -273.7798708315560816, -277.1557051578701021 ) ) ;
#34217=CARTESIAN_POINT ( 'NONE',  ( -34.26929567704836899, -296.2177434910190641, -343.6938585322489530 ) ) ;
#34218=CARTESIAN_POINT ( 'NONE',  ( -110.6838177606650220, -297.6531287954829281, -268.7397210085400729 ) ) ;
#34220=CARTESIAN_POINT ( 'NONE',  ( -93.09014237918928814, -297.4364882774215175, -322.3279147725669986 ) ) ;
#34221=CARTESIAN_POINT ( 'NONE',  ( -59.58077875099814236, -295.7647791030258304, -198.5054496197738843 ) ) ;
#34222=CARTESIAN_POINT ( 'NONE',  ( -25.40060182094608621, -292.8596558745691709, -198.1895098453764774 ) ) ;
#34223=CARTESIAN_POINT ( 'NONE',  ( -41.19492402420804211, -274.8077769369849648, -193.5671185644905847 ) ) ;
#34224=CARTESIAN_POINT ( 'NONE',  ( -110.9264423610149493, -289.1162361386358839, -271.1739069699857509 ) ) ;
#34226=CARTESIAN_POINT ( 'NONE',  ( -83.54814466294099873, -273.9300773406669123, -208.7762142314838911 ) ) ;
#34227=CARTESIAN_POINT ( 'NONE',  ( -109.3830825664299766, -296.7282134393302613, -282.2828084323656412 ) ) ;
#34228=CARTESIAN_POINT ( 'NONE',  ( 21.57323429183614039, -282.8890158616968051, -223.3572403919718852 ) ) ;
#34229=CARTESIAN_POINT ( 'NONE',  ( 39.21705108065572887, -280.2318014078542774, -269.9497440297685671 ) ) ;
#34230=CARTESIAN_POINT ( 'NONE',  ( -39.96779119002608383, -276.4328925534953783, -347.2273803231823877 ) ) ;
#34231=CARTESIAN_POINT ( 'NONE',  ( 38.81956285546804253, -279.9827276861665268, -272.7906105686262777 ) ) ;
#34232=CARTESIAN_POINT ( 'NONE',  ( 36.45962506064223874, -279.3692829259026098, -256.0995321736932624 ) ) ;
#34234=CARTESIAN_POINT ( 'NONE',  ( 20.32850651146596377, -273.4866402244899746, -224.6296565114017767 ) ) ;
#34235=CARTESIAN_POINT ( 'NONE',  ( -111.3752657656298624, -280.3942280740383808, -282.6731257642764490 ) ) ;
#34238=CARTESIAN_POINT ( 'NONE',  ( -88.90401600159579232, -295.5798497753087872, -214.4749743809273923 ) ) ;
#34239=CARTESIAN_POINT ( 'NONE',  ( 4.141534145870517492, -292.5943028513687523, -205.4277297367769961 ) ) ;
#34240=CARTESIAN_POINT ( 'NONE',  ( -41.26271802641029751, -279.1015408243997058, -345.4383451556131490 ) ) ;
#34241=CARTESIAN_POINT ( 'NONE',  ( -82.24870325765969881, -271.4397368065993419, -210.2263269272407626 ) ) ;
#34243=CARTESIAN_POINT ( 'NONE',  ( -6.029515109993660360, -284.5639764528982028, -339.1278342830471502 ) ) ;
#34245=CARTESIAN_POINT ( 'NONE',  ( 20.69450262605535329, -284.8969538493076925, -222.8355371794983739 ) ) ;
#34247=CARTESIAN_POINT ( 'NONE',  ( -26.16198268392631476, -293.7015660433197581, -342.9017577774432084 ) ) ;
#34248=CARTESIAN_POINT ( 'NONE',  ( 9.833386922018071630, -284.8494478140071919, -213.0429128530003595 ) ) ;
#34250=CARTESIAN_POINT ( 'NONE',  ( -48.10455602610596060, -293.1887845636665020, -344.6375315788861258 ) ) ;
#34251=CARTESIAN_POINT ( 'NONE',  ( -2.521853637551600968, -284.9840753035919079, -202.4474094002151787 ) ) ;
#34252=CARTESIAN_POINT ( 'NONE',  ( -52.00604184509451500, -281.4616148127890369, -197.9804177582704767 ) ) ;
#34253=CARTESIAN_POINT ( 'NONE',  ( -18.29566738581069529, -287.4972307677866183, -196.1088809619367623 ) ) ;
#34254=CARTESIAN_POINT ( 'NONE',  ( 35.21487320835912982, -279.5046721674019068, -247.7886196831189523 ) ) ;
#34255=CARTESIAN_POINT ( 'NONE',  ( 22.74990013573843584, -288.1296722827345889, -311.8319100754199553 ) ) ;
#34256=CARTESIAN_POINT ( 'NONE',  ( -35.66744503607664996, -281.4988063879697506, -196.7784320654212138 ) ) ;
#34257=CARTESIAN_POINT ( 'NONE',  ( -4.283733509695101027, -281.3022989234690385, -205.0802637488628193 ) ) ;
#34258=CARTESIAN_POINT ( 'NONE',  ( -49.11320288613227802, -287.8829048438245763, -195.8784366333053981 ) ) ;
#34260=CARTESIAN_POINT ( 'NONE',  ( -82.96886876072993289, -297.2806448308252811, -208.2693808175442030 ) ) ;
#34261=CARTESIAN_POINT ( 'NONE',  ( -112.0138432835007762, -292.5567814594156744, -268.4441217722098827 ) ) ;
#34263=CARTESIAN_POINT ( 'NONE',  ( -119.3990491898856732, -299.0519495502701943, -270.3937649182068412 ) ) ;
#34265=CARTESIAN_POINT ( 'NONE',  ( -70.56890234192968592, -271.6148902094227537, -202.9372241164959121 ) ) ;
#34267=CARTESIAN_POINT ( 'NONE',  ( -50.35119816610198740, -293.6153083487474760, -345.4957494738908963 ) ) ;
#34268=CARTESIAN_POINT ( 'NONE',  ( -108.6324653325803951, -272.1137697879979100, -254.1895545100026368 ) ) ;
#34269=CARTESIAN_POINT ( 'NONE',  ( -15.62906509933307042, -290.2863070416325968, -340.8365291625216287 ) ) ;
#34270=CARTESIAN_POINT ( 'NONE',  ( 36.70056719243410726, -283.2885614451192282, -268.5365362954483430 ) ) ;
#34271=CARTESIAN_POINT ( 'NONE',  ( -80.19502977914541475, -291.0449205970095363, -333.6879584039279507 ) ) ;
#34272=CARTESIAN_POINT ( 'NONE',  ( -113.6967297589361294, -291.9279614819956237, -265.5436786516995653 ) ) ;
#34273=CARTESIAN_POINT ( 'NONE',  ( -13.96619434067755350, -288.3554475984544752, -199.0424529753610159 ) ) ;
#34274=CARTESIAN_POINT ( 'NONE',  ( -64.74431301694771435, -279.8708442395716816, -198.3458938056077443 ) ) ;
#34275=CARTESIAN_POINT ( 'NONE',  ( -107.0560859384605976, -294.2527519572428787, -299.6379959025505286 ) ) ;
#34276=CARTESIAN_POINT ( 'NONE',  ( 23.40160874402737434, -282.0178754426440264, -317.7031431070628855 ) ) ;
#34277=CARTESIAN_POINT ( 'NONE',  ( 1.234442724714710504, -276.4336878167842428, -206.9359913965263615 ) ) ;
#34278=CARTESIAN_POINT ( 'NONE',  ( -102.0455923789670294, -275.4805209788415823, -239.2376011013261916 ) ) ;
#34279=CARTESIAN_POINT ( 'NONE',  ( 36.60053765842658891, -274.0145484192714775, -287.9247898054573511 ) ) ;
#34281=CARTESIAN_POINT ( 'NONE',  ( 22.63170659143023755, -281.6409211059499285, -312.0885541389795321 ) ) ;
#34282=CARTESIAN_POINT ( 'NONE',  ( -45.59152172870372510, -278.3594338719893244, -346.5712997914079665 ) ) ;
#34283=CARTESIAN_POINT ( 'NONE',  ( -12.76765362462998965, -285.4227241999366242, -197.6360435514263827 ) ) ;
#34284=CARTESIAN_POINT ( 'NONE',  ( -30.73858418250360458, -293.8969123540449573, -196.6429189189213105 ) ) ;
#34285=CARTESIAN_POINT ( 'NONE',  ( -104.9091053112616976, -274.6127828019201047, -235.0179643765321771 ) ) ;
#34286=CARTESIAN_POINT ( 'NONE',  ( -95.66270135784567685, -274.5392951448305894, -220.8236808529613882 ) ) ;
#34288=CARTESIAN_POINT ( 'NONE',  ( 35.64294824802102113, -275.3657226822650159, -268.8640856181839922 ) ) ;
#34289=CARTESIAN_POINT ( 'NONE',  ( -70.51442155949654023, -297.4907178355592237, -337.4401682410059493 ) ) ;
#34290=CARTESIAN_POINT ( 'NONE',  ( -98.84862977235592041, -283.1316085380729533, -227.7130625898168148 ) ) ;
#34291=CARTESIAN_POINT ( 'NONE',  ( -16.62822348594025712, -291.9794000890979646, -196.2214108288478940 ) ) ;
#34292=CARTESIAN_POINT ( 'NONE',  ( 10.70391374622207792, -274.4042966066276676, -327.4878699216591826 ) ) ;
#34293=CARTESIAN_POINT ( 'NONE',  ( -38.88334677667683081, -290.6713127872788505, -346.5455241523515042 ) ) ;
#34295=CARTESIAN_POINT ( 'NONE',  ( -106.8600781465329703, -289.7802122514539178, -247.0926588329597280 ) ) ;
#34297=CARTESIAN_POINT ( 'NONE',  ( 20.87341052307266409, -291.4542885754999588, -220.8476162752266703 ) ) ;
#34298=CARTESIAN_POINT ( 'NONE',  ( -108.3719724519020673, -289.9955164926557245, -287.2959312521699076 ) ) ;
#34300=CARTESIAN_POINT ( 'NONE',  ( 31.13957490063481259, -288.1857860432132838, -235.8385531977528728 ) ) ;
#34301=CARTESIAN_POINT ( 'NONE',  ( -105.5355565345349049, -279.2357093591211310, -244.1103662098799418 ) ) ;
#34303=CARTESIAN_POINT ( 'NONE',  ( 22.92021083850333341, -293.1096131384330761, -317.8162910149564482 ) ) ;
#34304=CARTESIAN_POINT ( 'NONE',  ( -30.90067008694625628, -286.7829176031515317, -193.7200004453037536 ) ) ;
#34305=CARTESIAN_POINT ( 'NONE',  ( -108.2060138686890269, -284.5010842381635712, -300.5639465899043330 ) ) ;
#34306=CARTESIAN_POINT ( 'NONE',  ( -33.49086671121882119, -283.3356625503565738, -343.2932290516056923 ) ) ;
#34307=CARTESIAN_POINT ( 'NONE',  ( 161.1277221853654567, 220.4622843307828362, -205.2806313236248172 ) ) ;
#34308=CARTESIAN_POINT ( 'NONE',  ( -96.32399440117350764, -238.8988692071569346, -340.6895823940229207 ) ) ;
#34309=CARTESIAN_POINT ( 'NONE',  ( -110.6513661324959799, -268.1078488974698075, -295.2803869936869887 ) ) ;
#34310=CARTESIAN_POINT ( 'NONE',  ( 33.01813753705873467, -274.4826219557081117, -250.1276976304746995 ) ) ;
#34311=CARTESIAN_POINT ( 'NONE',  ( 28.30119289759938539, -274.9145425739268376, -303.1134761622107590 ) ) ;
#34312=CARTESIAN_POINT ( 'NONE',  ( -43.27874660773018434, -297.4868686218536027, -193.5989001875758220 ) ) ;
#34313=CARTESIAN_POINT ( 'NONE',  ( -61.73251378320581750, -183.4071649071924242, -359.1965488161292797 ) ) ;
#34314=CARTESIAN_POINT ( 'NONE',  ( 38.00935004060875855, -274.0692830204630468, -257.0378656803317767 ) ) ;
#34315=CARTESIAN_POINT ( 'NONE',  ( -88.04357619820882519, -275.0916577905791200, -216.3715997071691675 ) ) ;
#34316=CARTESIAN_POINT ( 'NONE',  ( -22.69223961301342030, -293.3237631074124465, -198.5306273864514992 ) ) ;
#34318=CARTESIAN_POINT ( 'NONE',  ( -113.3703997158275314, -297.6276267735301531, -259.6613486210976589 ) ) ;
#34319=CARTESIAN_POINT ( 'NONE',  ( 34.07216301272951142, -288.2485867149433147, -285.8486415548811692 ) ) ;
#34320=CARTESIAN_POINT ( 'NONE',  ( -74.51925168996828575, -296.3361975368093226, -337.6664339425890375 ) ) ;
#34321=CARTESIAN_POINT ( 'NONE',  ( -72.04066619508130032, -295.9910215724125919, -339.0306793425191927 ) ) ;
#34322=CARTESIAN_POINT ( 'NONE',  ( 14.87402335077873694, -292.9800392262783362, -219.2738369918496346 ) ) ;
#34324=CARTESIAN_POINT ( 'NONE',  ( 8.614788117518424215, -276.5964915159101452, -210.3834939606303465 ) ) ;
#34326=CARTESIAN_POINT ( 'NONE',  ( -36.74672813071549626, -279.5670981175811676, -193.4119214969759071 ) ) ;
#34329=CARTESIAN_POINT ( 'NONE',  ( 7.734620083320801420, -277.3608841345051701, -328.1451861399400514 ) ) ;
#34330=CARTESIAN_POINT ( 'NONE',  ( -4.287439431814018320, -276.2419815574499466, -201.9261198778575874 ) ) ;
#34331=CARTESIAN_POINT ( 'NONE',  ( -56.53007240974637426, -275.3182346430110670, -343.2862094483174928 ) ) ;
#34332=CARTESIAN_POINT ( 'NONE',  ( -66.86810800618894746, -298.3061433685239194, -203.4737768698030322 ) ) ;
#34333=CARTESIAN_POINT ( 'NONE',  ( -105.2994578507293966, -295.5024658064982077, -242.1278383106127876 ) ) ;
#34335=CARTESIAN_POINT ( 'NONE',  ( 3.783775467739847631, -281.0818629129884698, -205.2734087682872826 ) ) ;
#34336=CARTESIAN_POINT ( 'NONE',  ( 32.51700731755104101, -275.9998503382088870, -291.5884344696497692 ) ) ;
#34337=CARTESIAN_POINT ( 'NONE',  ( 95.12341659969116847, -301.7069487475465053, -195.1494023596418401 ) ) ;
#34339=CARTESIAN_POINT ( 'NONE',  ( 25.09383745451428993, -286.2250496370473343, -232.2244509347945325 ) ) ;
#34340=CARTESIAN_POINT ( 'NONE',  ( 9.940883578797246045, -278.9533739524090379, -213.3528190261110353 ) ) ;
#34341=CARTESIAN_POINT ( 'NONE',  ( -62.49341625694517433, -278.2932417685403834, -201.1497904846716551 ) ) ;
#34342=CARTESIAN_POINT ( 'NONE',  ( -67.15838207566098106, -281.5259498496460537, -338.5825810328841499 ) ) ;
#34343=CARTESIAN_POINT ( 'NONE',  ( 36.36333724091495867, -289.3707106050999300, -256.2159359082284595 ) ) ;
#34344=CARTESIAN_POINT ( 'NONE',  ( -54.02937501091456340, -278.4761517153036721, -341.8883748483089562 ) ) ;
#34346=CARTESIAN_POINT ( 'NONE',  ( -1.775349572001520437, -294.5235961200840507, -204.3305541583093259 ) ) ;
#34347=CARTESIAN_POINT ( 'NONE',  ( -31.55016583279567044, -275.2199800603388553, -346.1786885303034751 ) ) ;
#34348=CARTESIAN_POINT ( 'NONE',  ( 33.68754545615291107, -276.4319247689645067, -287.6979399312593841 ) ) ;
#34349=CARTESIAN_POINT ( 'NONE',  ( 30.74286868156538333, -283.9714973105206468, -302.3353627035035061 ) ) ;
#34353=CARTESIAN_POINT ( 'NONE',  ( -41.65347839045332989, -291.0261908240518096, -345.8109723246171825 ) ) ;
#34354=CARTESIAN_POINT ( 'NONE',  ( -109.3542225294415431, -294.8223437452031135, -249.3586537272184955 ) ) ;
#34355=CARTESIAN_POINT ( 'NONE',  ( -112.8376330404410623, -283.9319766955698014, -255.7833246669176788 ) ) ;
#34357=CARTESIAN_POINT ( 'NONE',  ( -31.28246849525034889, -272.8150698232893774, -197.1054365290772807 ) ) ;
#34358=CARTESIAN_POINT ( 'NONE',  ( 32.97861392227385124, -291.3790443439824571, -246.4118958209336085 ) ) ;
#34361=CARTESIAN_POINT ( 'NONE',  ( -106.6227382823926888, -289.4463189894174207, -238.2533404958382448 ) ) ;
#34362=CARTESIAN_POINT ( 'NONE',  ( -96.55153093812802467, -285.5410322633265991, -314.4137722981006391 ) ) ;
#34363=CARTESIAN_POINT ( 'NONE',  ( 22.21187373955070399, -285.1518710447642206, -223.1456054474440691 ) ) ;
#34364=CARTESIAN_POINT ( 'NONE',  ( -93.71811311218314700, -286.6436815332673973, -223.0633910003248559 ) ) ;
#34365=CARTESIAN_POINT ( 'NONE',  ( -79.41047151466197818, -286.2709442036873497, -210.4422534570611276 ) ) ;
#34366=CARTESIAN_POINT ( 'NONE',  ( -110.0525177619899608, -292.7858430085201462, -250.5246275286232560 ) ) ;
#34367=CARTESIAN_POINT ( 'NONE',  ( 38.11783618578413524, -273.5707590769894750, -265.5561813837308591 ) ) ;
#34368=CARTESIAN_POINT ( 'NONE',  ( 37.26368665711515860, -275.6480175737946183, -251.3932358063823926 ) ) ;
#34369=CARTESIAN_POINT ( 'NONE',  ( 20.22945842752876189, -290.9594868272411077, -221.4038739008998391 ) ) ;
#34370=CARTESIAN_POINT ( 'NONE',  ( -112.1751809025142563, -278.3246334919494416, -288.5533267873198611 ) ) ;
#34371=CARTESIAN_POINT ( 'NONE',  ( -89.63657740796014650, -297.7733496304020377, -323.6980982053268576 ) ) ;
#34374=CARTESIAN_POINT ( 'NONE',  ( -99.45674586159880448, -282.6966867225173132, -309.7370110110442170 ) ) ;
#34375=CARTESIAN_POINT ( 'NONE',  ( -105.5883585953012300, -276.9616102259463446, -239.1332106464525395 ) ) ;
#34377=CARTESIAN_POINT ( 'NONE',  ( 38.62899887940997701, -273.9349658006638606, -262.6696517351882108 ) ) ;
#34378=CARTESIAN_POINT ( 'NONE',  ( -29.71102177160464919, -276.3017135885889388, -343.1146765248514612 ) ) ;
#34379=CARTESIAN_POINT ( 'NONE',  ( -31.52853196405320446, -296.4976994272366824, -343.8754043053045848 ) ) ;
#34380=CARTESIAN_POINT ( 'NONE',  ( 26.03297098550137534, -279.8995512609359366, -227.0811265355436319 ) ) ;
#34381=CARTESIAN_POINT ( 'NONE',  ( 14.49125631696822758, -295.2424324232451909, -322.1697811389622643 ) ) ;
#34382=CARTESIAN_POINT ( 'NONE',  ( -69.30652115517672485, -296.7791327756492024, -339.8847979521177649 ) ) ;
#34383=CARTESIAN_POINT ( 'NONE',  ( -34.47780499870007986, -297.9223065719783676, -197.3612017988505727 ) ) ;
#34384=CARTESIAN_POINT ( 'NONE',  ( -111.2520230561674595, -292.7196854557986399, -257.3257027662428982 ) ) ;
#34385=CARTESIAN_POINT ( 'NONE',  ( -95.81795164386677754, -285.3954585061459852, -220.1859557684366848 ) ) ;
#34386=CARTESIAN_POINT ( 'NONE',  ( 27.45859864681588647, -273.1698047327267886, -231.0023116163505108 ) ) ;
#34387=CARTESIAN_POINT ( 'NONE',  ( -6.921879216600030027, -288.4971779233227380, -341.1117311504117424 ) ) ;
#34388=CARTESIAN_POINT ( 'NONE',  ( -19.15774003294121286, -282.2670616715863048, -197.9115887071694715 ) ) ;
#34389=CARTESIAN_POINT ( 'NONE',  ( -83.78787137941044705, -284.4553066762796902, -213.6722582427379677 ) ) ;
#34390=CARTESIAN_POINT ( 'NONE',  ( -15.55813322307565016, -286.7702195599200081, -342.1822380205039735 ) ) ;
#34391=CARTESIAN_POINT ( 'NONE',  ( 168.8235619055982113, 230.3815547064285738, -190.2228674158758395 ) ) ;
#34392=CARTESIAN_POINT ( 'NONE',  ( 35.74209824558113979, -287.0328589921418256, -268.3169883584774880 ) ) ;
#34394=CARTESIAN_POINT ( 'NONE',  ( -35.89158398408883954, -283.9756625876280509, -347.1252036715262079 ) ) ;
#34395=CARTESIAN_POINT ( 'NONE',  ( -113.1296680739815486, -289.4577737145420997, -282.5678426761463129 ) ) ;
#34396=CARTESIAN_POINT ( 'NONE',  ( -110.6651107440872579, -279.8896169866504806, -291.1004012884798726 ) ) ;
#34397=CARTESIAN_POINT ( 'NONE',  ( -108.0632179359445217, -280.2406374262168924, -241.1761014407339303 ) ) ;
#34398=CARTESIAN_POINT ( 'NONE',  ( 25.13738525290967019, -280.8646270068728654, -232.5091624251931819 ) ) ;
#34399=CARTESIAN_POINT ( 'NONE',  ( -27.03999911022992464, -276.1831539452681454, -196.0196911955375185 ) ) ;
#34400=CARTESIAN_POINT ( 'NONE',  ( -81.87170042775603918, -295.6400822892362044, -333.2440651155099545 ) ) ;
#34401=CARTESIAN_POINT ( 'NONE',  ( -80.46073557092442741, -289.4850982609135031, -209.3667043154135570 ) ) ;
#34402=CARTESIAN_POINT ( 'NONE',  ( -105.0424347250891088, -295.8480110624270196, -242.2393006899522732 ) ) ;
#34405=CARTESIAN_POINT ( 'NONE',  ( 1.880424467474606232, -284.4435518456094201, -333.6901038841115792 ) ) ;
#34406=CARTESIAN_POINT ( 'NONE',  ( -108.1944290656878138, -296.4524985918720859, -252.6470326448538231 ) ) ;
#34407=CARTESIAN_POINT ( 'NONE',  ( -11.27131494089022112, -293.4635790433106308, -198.1816136454255002 ) ) ;
#34408=CARTESIAN_POINT ( 'NONE',  ( -92.63079257372240249, -284.5229192956703059, -318.2028465473765095 ) ) ;
#34409=CARTESIAN_POINT ( 'NONE',  ( 1.088043482133245643, -273.6107938251679457, -203.8930754212499323 ) ) ;
#34410=CARTESIAN_POINT ( 'NONE',  ( -112.1615808059637516, -290.9804904538661390, -288.1740737290444940 ) ) ;
#34411=CARTESIAN_POINT ( 'NONE',  ( -77.84185929621585842, -283.6538506491528437, -206.3295430632726379 ) ) ;
#34412=CARTESIAN_POINT ( 'NONE',  ( -90.77431561969035556, -291.6527652021401877, -214.8732379378299697 ) ) ;
#34413=CARTESIAN_POINT ( 'NONE',  ( 29.97961654823861011, -287.5044664644527188, -241.9471960021442669 ) ) ;
#34416=CARTESIAN_POINT ( 'NONE',  ( 121.5961377311245286, 147.4458027207525959, -260.2603503459518492 ) ) ;
#34417=CARTESIAN_POINT ( 'NONE',  ( -52.75843894939779943, -284.7662221351927769, -345.1481875036043334 ) ) ;
#34418=CARTESIAN_POINT ( 'NONE',  ( -69.91165696735023971, -280.9809262143061233, -337.9199732462171255 ) ) ;
#34420=CARTESIAN_POINT ( 'NONE',  ( 35.44498595126895424, -280.5926609329131338, -279.5103997065099861 ) ) ;
#34421=CARTESIAN_POINT ( 'NONE',  ( 36.47198018288536048, -275.4935564024168002, -292.2544667241347724 ) ) ;
#34422=CARTESIAN_POINT ( 'NONE',  ( -108.8614118121294183, -280.2657354845103441, -292.5562303587832389 ) ) ;
#34423=CARTESIAN_POINT ( 'NONE',  ( 191.0641345987445163, 268.5554630237342622, -138.4309074710560310 ) ) ;
#34424=CARTESIAN_POINT ( 'NONE',  ( 31.49856704163147469, -279.6968260851338073, -237.0787524178924741 ) ) ;
#34425=CARTESIAN_POINT ( 'NONE',  ( -111.9526466618658986, -282.6012555446652073, -268.1131284285407901 ) ) ;
#34426=CARTESIAN_POINT ( 'NONE',  ( -99.17073380490339218, -297.7183258460046886, -314.6214715509760254 ) ) ;
#34427=CARTESIAN_POINT ( 'NONE',  ( 33.17774435946422074, -294.2972247446610368, -289.5135801892748759 ) ) ;
#34430=CARTESIAN_POINT ( 'NONE',  ( -92.02899275269409429, -289.9351381479788756, -221.2450139474152309 ) ) ;
#34431=CARTESIAN_POINT ( 'NONE',  ( 3.454464988765484357, -277.1707214683469260, -335.6080471256983060 ) ) ;
#34432=CARTESIAN_POINT ( 'NONE',  ( -44.57119715687876038, -298.1249496152082656, -197.6696018032382085 ) ) ;
#34434=CARTESIAN_POINT ( 'NONE',  ( -111.5157528953660773, -271.7197193927910348, -250.6720555277861422 ) ) ;
#34438=CARTESIAN_POINT ( 'NONE',  ( 35.01084741140333989, -282.7868857179768725, -282.1651401161536796 ) ) ;
#34439=CARTESIAN_POINT ( 'NONE',  ( -45.19128283315919248, -281.7143077829297226, -194.7286812767119102 ) ) ;
#34440=CARTESIAN_POINT ( 'NONE',  ( -93.61052407174892664, -282.9479289194104581, -317.2357155893429308 ) ) ;
#34441=CARTESIAN_POINT ( 'NONE',  ( 5.619022418208107439, -282.5014833054891028, -209.8198775243695025 ) ) ;
#34442=CARTESIAN_POINT ( 'NONE',  ( 30.91294705439283064, -274.4023282231539156, -298.2818951294642602 ) ) ;
#34445=CARTESIAN_POINT ( 'NONE',  ( -84.75868227401930710, -278.4894663070232355, -330.8918373463444595 ) ) ;
#34449=CARTESIAN_POINT ( 'NONE',  ( -108.8199239636463886, -286.7346503857783659, -245.2380410084283255 ) ) ;
#34450=CARTESIAN_POINT ( 'NONE',  ( 25.92719344400298809, -293.2522292200643506, -307.0986850329196045 ) ) ;
#34451=CARTESIAN_POINT ( 'NONE',  ( 34.97377452075691195, -287.2331697622225306, -296.6652753883899436 ) ) ;
#34452=CARTESIAN_POINT ( 'NONE',  ( -38.62023927312097982, -284.2757960434743154, -196.3461698476520496 ) ) ;
#34453=CARTESIAN_POINT ( 'NONE',  ( -81.82041076653520406, -284.0072811204997265, -211.7350212728857173 ) ) ;
#34454=CARTESIAN_POINT ( 'NONE',  ( -29.08198625561179540, -287.1858934527450060, -343.9121284406027712 ) ) ;
#34455=CARTESIAN_POINT ( 'NONE',  ( -76.32509074125809434, -284.7907593140988638, -332.6098479994429908 ) ) ;
#34456=CARTESIAN_POINT ( 'NONE',  ( -28.85336403914640258, -274.9445047084882390, -344.9314109430496842 ) ) ;
#34458=CARTESIAN_POINT ( 'NONE',  ( -40.75997245557036308, -284.4098419713503176, -194.1861727472378618 ) ) ;
#34459=CARTESIAN_POINT ( 'NONE',  ( -88.26942142089335164, -299.3395460229289142, -215.2328837326363384 ) ) ;
#34460=CARTESIAN_POINT ( 'NONE',  ( -90.58595351819140262, -283.2996294840405085, -217.3038102252114641 ) ) ;
#34461=CARTESIAN_POINT ( 'NONE',  ( 35.92247115567383275, -282.4698039833236294, -268.5658872690150929 ) ) ;
#34462=CARTESIAN_POINT ( 'NONE',  ( 37.77361692184092590, -289.6027893320435282, -274.3008295043401290 ) ) ;
#34467=CARTESIAN_POINT ( 'NONE',  ( -14.19939524585035961, -296.6744614328374041, -342.2898877545442247 ) ) ;
#34468=CARTESIAN_POINT ( 'NONE',  ( -54.93796967040349699, -277.8258897703540811, -197.4008982300556454 ) ) ;
#34469=CARTESIAN_POINT ( 'NONE',  ( -90.66649956086934026, -290.5168344573802415, -214.9643708368327282 ) ) ;
#34470=CARTESIAN_POINT ( 'NONE',  ( -0.3746848051724631090, -292.9521636844906425, -334.2933756579137707 ) ) ;
#34471=CARTESIAN_POINT ( 'NONE',  ( -57.23068963013539445, -278.4749008588608490, -199.6103471502528635 ) ) ;
#34472=CARTESIAN_POINT ( 'NONE',  ( -40.54800285653801950, -296.1510210072717655, -196.1824271889297790 ) ) ;
#34473=CARTESIAN_POINT ( 'NONE',  ( 21.37779253009841085, -294.2508382499786990, -226.1653641004419057 ) ) ;
#34474=CARTESIAN_POINT ( 'NONE',  ( 10.64812456238589888, -290.9090924074130839, -330.4860931364851808 ) ) ;
#34475=CARTESIAN_POINT ( 'NONE',  ( -113.2554394086487122, -294.9344315055139987, -278.0949359362051609 ) ) ;
#34476=CARTESIAN_POINT ( 'NONE',  ( -48.15832248838597707, -290.7920557362944578, -343.4157190178026440 ) ) ;
#34477=CARTESIAN_POINT ( 'NONE',  ( 20.55313342022535039, -291.1194737908845127, -221.1257645571029968 ) ) ;
#34478=CARTESIAN_POINT ( 'NONE',  ( -109.9979881531174186, -291.8235393901262569, -282.1209556693643776 ) ) ;
#34480=CARTESIAN_POINT ( 'NONE',  ( -96.89875502240515459, -291.9483574705202500, -227.7835419696766621 ) ) ;
#34482=CARTESIAN_POINT ( 'NONE',  ( 128.9467878515196162, -299.5541904835127980, -191.8695490883551713 ) ) ;
#34483=CARTESIAN_POINT ( 'NONE',  ( -113.4173267146450428, -291.6389339432477072, -279.7708067382703234 ) ) ;
#34484=CARTESIAN_POINT ( 'NONE',  ( 16.07534854567625615, -278.8247427304797839, -217.1369527966763258 ) ) ;
#34485=CARTESIAN_POINT ( 'NONE',  ( 33.77542244239630520, -293.7701131912468213, -286.8890402137017759 ) ) ;
#34486=CARTESIAN_POINT ( 'NONE',  ( 36.59971959299395650, -281.2821715439123977, -248.8274243594463258 ) ) ;
#34487=CARTESIAN_POINT ( 'NONE',  ( -41.57222159324769706, -282.7706467632410181, -347.2759500177445489 ) ) ;
#34488=CARTESIAN_POINT ( 'NONE',  ( 20.92532150693828186, -286.1996689714279682, -317.3183604583745705 ) ) ;
#34489=CARTESIAN_POINT ( 'NONE',  ( 6.299435604253456056, -280.5919680786410026, -330.4137344928267908 ) ) ;
#34490=CARTESIAN_POINT ( 'NONE',  ( -18.65505521339254358, -284.2925103443244552, -197.6726712581372283 ) ) ;
#34492=CARTESIAN_POINT ( 'NONE',  ( -45.18269783257633065, -278.4345733944429071, -194.4058613743342789 ) ) ;
#34493=CARTESIAN_POINT ( 'NONE',  ( -63.08467999146868976, -284.6449058034670543, -198.1199143853961857 ) ) ;
#34495=CARTESIAN_POINT ( 'NONE',  ( -19.90266939806262769, -293.8800543272038226, -198.5983034260257796 ) ) ;
#34496=CARTESIAN_POINT ( 'NONE',  ( -21.49484026384161695, -275.6767900491931869, -195.6116475915521278 ) ) ;
#34497=CARTESIAN_POINT ( 'NONE',  ( -56.60983698365105710, -276.9740435781957899, -340.8467662633546524 ) ) ;
#34498=CARTESIAN_POINT ( 'NONE',  ( -113.8132956795790278, -290.6007056543592171, -279.8063793833225645 ) ) ;
#34499=CARTESIAN_POINT ( 'NONE',  ( -60.80812581265943351, -281.4340131131065164, -342.2394482817100538 ) ) ;
#34500=CARTESIAN_POINT ( 'NONE',  ( -95.29325446982903713, -290.2393239521967416, -225.5836035559018171 ) ) ;
#34501=CARTESIAN_POINT ( 'NONE',  ( -94.99089284043095915, -293.8893466730493742, -318.3557897135404460 ) ) ;
#34504=CARTESIAN_POINT ( 'NONE',  ( 10.97619768048102173, -292.2496508454993887, -215.4905999240959034 ) ) ;
#34506=CARTESIAN_POINT ( 'NONE',  ( 17.36665895637873192, -279.6952119285918457, -314.0302885647153062 ) ) ;
#34507=CARTESIAN_POINT ( 'NONE',  ( -99.72332902484235717, -296.2055648554388085, -225.6246385783369419 ) ) ;
#34508=CARTESIAN_POINT ( 'NONE',  ( 12.20262674270734671, -278.8726780447990450, -213.0403961371587798 ) ) ;
#34509=CARTESIAN_POINT ( 'NONE',  ( -107.4807738000744024, -286.2608951435111635, -239.6703052914083969 ) ) ;
#34510=CARTESIAN_POINT ( 'NONE',  ( 27.65910688053578426, -286.9327292443600754, -237.0247421569294204 ) ) ;
#34511=CARTESIAN_POINT ( 'NONE',  ( -5.963997703303300923, -278.1521721042677200, -337.0544580163593764 ) ) ;
#34512=CARTESIAN_POINT ( 'NONE',  ( -53.53011605969862075, -293.2808115628807286, -343.2825283670604790 ) ) ;
#34513=CARTESIAN_POINT ( 'NONE',  ( -94.71401309191251983, -297.6592379747346513, -317.1398977948419429 ) ) ;
#34514=CARTESIAN_POINT ( 'NONE',  ( -59.32848412113337133, -276.1381511209346513, -340.3876260613907334 ) ) ;
#34517=CARTESIAN_POINT ( 'NONE',  ( -111.9492066669793502, -295.9809642571930794, -289.3738872927775105 ) ) ;
#34518=CARTESIAN_POINT ( 'NONE',  ( -12.79032193891064750, -290.6506754433610240, -340.6358931573682867 ) ) ;
#34520=CARTESIAN_POINT ( 'NONE',  ( 20.44313945308228497, -288.8334891937228690, -315.1564373390917808 ) ) ;
#34522=CARTESIAN_POINT ( 'NONE',  ( -67.25966938265867157, -278.7280572067947446, -199.6664553196427789 ) ) ;
#34523=CARTESIAN_POINT ( 'NONE',  ( -92.61796089930656706, -296.4702183842724708, -323.8199599234287120 ) ) ;
#34524=CARTESIAN_POINT ( 'NONE',  ( -106.6118312258548286, -288.2922316099459863, -301.1815219726607893 ) ) ;
#34525=CARTESIAN_POINT ( 'NONE',  ( -101.6082741705620975, -296.3270059421107590, -312.8314635531399972 ) ) ;
#34526=CARTESIAN_POINT ( 'NONE',  ( 30.60679580778791475, -294.2445842736326540, -297.2406384185550223 ) ) ;
#34529=CARTESIAN_POINT ( 'NONE',  ( 25.29378254256534220, -289.6544581035109900, -314.0351727633541827 ) ) ;
#34530=CARTESIAN_POINT ( 'NONE',  ( -37.30987171927208124, -285.5519495502701375, -350.3611179825600175 ) ) ;
#34531=CARTESIAN_POINT ( 'NONE',  ( 39.42683758538345984, -280.9671249108991447, -275.6621480945013332 ) ) ;
#34532=CARTESIAN_POINT ( 'NONE',  ( -110.2046653653369219, -286.3321290529585781, -287.4762342893231448 ) ) ;
#34533=CARTESIAN_POINT ( 'NONE',  ( 38.99009174591972737, -286.0702963164138168, -265.8712515919215207 ) ) ;
#34534=CARTESIAN_POINT ( 'NONE',  ( -111.6822158206867499, -288.6933252414446542, -265.6200073272600548 ) ) ;
#34535=CARTESIAN_POINT ( 'NONE',  ( 5.197654779962012306, -278.3438286377333952, -333.0564827436386395 ) ) ;
#34537=CARTESIAN_POINT ( 'NONE',  ( -89.08582096261814343, -277.8045655973551789, -321.9260632020282742 ) ) ;
#34538=CARTESIAN_POINT ( 'NONE',  ( 34.32897561111584395, -281.0911912937279453, -284.8187613819188755 ) ) ;
#34539=CARTESIAN_POINT ( 'NONE',  ( 27.39531376834699472, -277.1739786188628045, -311.5769053578295029 ) ) ;
#34540=CARTESIAN_POINT ( 'NONE',  ( -86.53790579271186800, -278.1814631050417574, -211.5745152597847039 ) ) ;
#34541=CARTESIAN_POINT ( 'NONE',  ( -112.4526163206608231, -268.5066740142938215, -295.6311755849135352 ) ) ;
#34542=CARTESIAN_POINT ( 'NONE',  ( -55.29026660099994928, -274.7679486200987640, -195.7242023586695439 ) ) ;
#34543=CARTESIAN_POINT ( 'NONE',  ( -40.43472329958058253, -299.4393855005943692, -193.9612445427866305 ) ) ;
#34544=CARTESIAN_POINT ( 'NONE',  ( 35.78497577281001440, -290.2662352645559167, -287.0191576251351080 ) ) ;
#34546=CARTESIAN_POINT ( 'NONE',  ( 82.67471867677929254, -297.5265350176030097, -193.8629188578358082 ) ) ;
#34547=CARTESIAN_POINT ( 'NONE',  ( 32.96252191058563596, -288.3575734522253811, -249.5432643330654230 ) ) ;
#34548=CARTESIAN_POINT ( 'NONE',  ( 23.04234736230505831, -288.6888163792721116, -224.2123508952122108 ) ) ;
#34549=CARTESIAN_POINT ( 'NONE',  ( 35.75703090533297512, -286.9097485042926792, -271.0453614559516495 ) ) ;
#34550=CARTESIAN_POINT ( 'NONE',  ( -110.6288418090038590, -283.7646319219435327, -293.8251174885087380 ) ) ;
#34551=CARTESIAN_POINT ( 'NONE',  ( -68.84651728064750387, -278.0307267494371786, -203.6236703702743682 ) ) ;
#34552=CARTESIAN_POINT ( 'NONE',  ( -90.56469338685171522, -287.1490864046858746, -218.5362054788905368 ) ) ;
#34553=CARTESIAN_POINT ( 'NONE',  ( 35.16416309713526545, -280.2051275255844871, -283.6077479225878619 ) ) ;
#34554=CARTESIAN_POINT ( 'NONE',  ( -110.6590162693105697, -279.7916875897342379, -276.1341863933739660 ) ) ;
#34555=CARTESIAN_POINT ( 'NONE',  ( 5.437890585134830701, -276.9480443106114649, -329.6510820946421632 ) ) ;
#34556=CARTESIAN_POINT ( 'NONE',  ( -54.42805809455079924, -288.0617348201380423, -345.0886046087621253 ) ) ;
#34557=CARTESIAN_POINT ( 'NONE',  ( 13.58143929551368956, -283.1633392131408868, -327.9731760200120902 ) ) ;
#34558=CARTESIAN_POINT ( 'NONE',  ( -114.2792590192606639, -285.0491637650850407, -269.9883782335236333 ) ) ;
#34559=CARTESIAN_POINT ( 'NONE',  ( 25.56010813453520569, -282.2288590907139110, -307.5064218809916383 ) ) ;
#34563=CARTESIAN_POINT ( 'NONE',  ( -78.93641302016149552, -293.3587105215989936, -206.9723678381691343 ) ) ;
#34564=CARTESIAN_POINT ( 'NONE',  ( -27.89327738334935702, -290.8544169359388434, -194.3866062035648667 ) ) ;
#34565=CARTESIAN_POINT ( 'NONE',  ( -6.418763196234174906, -273.5273567616102923, -203.9745197839474429 ) ) ;
#34567=CARTESIAN_POINT ( 'NONE',  ( 35.38729568571260131, -293.2177794617452378, -295.5003503322957386 ) ) ;
#34568=CARTESIAN_POINT ( 'NONE',  ( -50.89782268737861415, -287.7082314833911028, -342.8490499431250669 ) ) ;
#34569=CARTESIAN_POINT ( 'NONE',  ( 36.43273151372589069, -291.8693157479862066, -276.3031081989711311 ) ) ;
#34570=CARTESIAN_POINT ( 'NONE',  ( -97.66655934481302381, -291.1775800709074247, -312.1927829385695077 ) ) ;
#34572=CARTESIAN_POINT ( 'NONE',  ( -107.6092279252722079, -292.8944583273994340, -243.9932327443221141 ) ) ;
#34573=CARTESIAN_POINT ( 'NONE',  ( -71.32018443880221525, -289.6044789259737513, -203.2984452164165532 ) ) ;
#34574=CARTESIAN_POINT ( 'NONE',  ( 13.18031646314293326, -294.7580393374967684, -214.8612865770728320 ) ) ;
#34575=CARTESIAN_POINT ( 'NONE',  ( -62.65541679911248707, -286.6558475602777776, -201.5856806804226267 ) ) ;
#34576=CARTESIAN_POINT ( 'NONE',  ( 21.65294137701133437, -294.9138446617339469, -223.7609429230506350 ) ) ;
#34579=CARTESIAN_POINT ( 'NONE',  ( 14.86887508249319367, -276.7636118066307631, -216.0245498427186703 ) ) ;
#34580=CARTESIAN_POINT ( 'NONE',  ( -64.21929981884952099, -294.5912615907673171, -342.3455152867368270 ) ) ;
#34581=CARTESIAN_POINT ( 'NONE',  ( 36.02794479340695943, -273.6652770988968086, -260.6210349547996543 ) ) ;
#34582=CARTESIAN_POINT ( 'NONE',  ( -109.3596389534653781, -276.8764407357224400, -251.4768180969392120 ) ) ;
#34583=CARTESIAN_POINT ( 'NONE',  ( -65.98216440058961041, -274.8738942027691223, -202.7826131767733386 ) ) ;
#34584=CARTESIAN_POINT ( 'NONE',  ( -2.807483554621384769, -273.0743087580672182, -202.1849961944236043 ) ) ;
#34586=CARTESIAN_POINT ( 'NONE',  ( -71.18576188694183315, -296.9332812589670993, -335.7201018960165015 ) ) ;
#34587=FACE_OUTER_BOUND ( 'NONE', #81554, .T. ) ;
#34588=CARTESIAN_POINT ( 'NONE',  ( -90.16952861421962950, -298.0844593871178176, -219.6741583514998126 ) ) ;
#34590=CARTESIAN_POINT ( 'NONE',  ( 25.01086344563809405, -285.0019460666180748, -228.0229928986286438 ) ) ;
#34591=CARTESIAN_POINT ( 'NONE',  ( -71.66500064822257343, -297.5853211811107144, -205.9193558477847148 ) ) ;
#34592=CARTESIAN_POINT ( 'NONE',  ( -15.41345741595617191, -286.3282382084300366, -196.4941265103896342 ) ) ;
#34593=CARTESIAN_POINT ( 'NONE',  ( 3.165398693109778616, -288.1908857818256138, -335.8829412456078103 ) ) ;
#34594=CARTESIAN_POINT ( 'NONE',  ( -98.65518058094846765, -297.9380413146176352, -314.2560900600401510 ) ) ;
#34595=CARTESIAN_POINT ( 'NONE',  ( -61.63173961456090666, -293.3681722867557369, -341.1975567680864287 ) ) ;
#34596=CARTESIAN_POINT ( 'NONE',  ( 38.63663579299326045, -280.6013040200209616, -258.5505073246328038 ) ) ;
#34597=CARTESIAN_POINT ( 'NONE',  ( 10.64812456238590599, -290.1952119285919593, -210.2361428286349394 ) ) ;
#34599=CARTESIAN_POINT ( 'NONE',  ( -94.42272174201055179, -288.6980192964061303, -316.5009866179692040 ) ) ;
#34600=DIRECTION ( 'NONE',  ( 0.000000000000000000, 0.000000000000000000, -1.000000000000000000 ) ) ;
#34601=CARTESIAN_POINT ( 'NONE',  ( -0.01766084105187968809, -286.5557158181418345, -335.4740706220597417 ) ) ;
#34602=CARTESIAN_POINT ( 'NONE',  ( -65.90091281252909994, -299.2722726813432814, -202.3110497454203767 ) ) ;
#34603=CARTESIAN_POINT ( 'NONE',  ( -42.40923899826706389, -281.4146846008261491, -194.1185685564796302 ) ) ;
#34604=CARTESIAN_POINT ( 'NONE',  ( -110.6678946213038301, -294.7942415013578739, -252.9922950953641418 ) ) ;
#34605=CARTESIAN_POINT ( 'NONE',  ( 31.97660595615275270, -281.2463814598186218, -247.3113535767344047 ) ) ;
#34606=CARTESIAN_POINT ( 'NONE',  ( -107.7738903629742993, -297.1173305717759945, -239.1116573494658439 ) ) ;
#34607=CARTESIAN_POINT ( 'NONE',  ( -60.75434593138362516, -299.2630604455569596, -200.4318485855384893 ) ) ;
#34608=CARTESIAN_POINT ( 'NONE',  ( 22.14502174142588586, -282.9264981027533281, -224.6637787299186755 ) ) ;
#34610=CARTESIAN_POINT ( 'NONE',  ( -72.04195674896796220, -272.5025988883462560, -205.7281070642440568 ) ) ;
#34612=CARTESIAN_POINT ( 'NONE',  ( -94.66946032890704998, -285.8686005303220554, -318.1667109234761028 ) ) ;
#34614=CARTESIAN_POINT ( 'NONE',  ( -55.63300648810263738, -280.7666405000205145, -350.3538533559490702 ) ) ;
#34615=CARTESIAN_POINT ( 'NONE',  ( -5.361322481310194732, -275.8391315646637167, -340.2282366200897741 ) ) ;
#34617=CARTESIAN_POINT ( 'NONE',  ( 14.87699211465616322, -292.6467328876990450, -219.2768713194639645 ) ) ;
#34618=CARTESIAN_POINT ( 'NONE',  ( -18.54023596828037057, -284.3258151337365689, -341.6685865295860935 ) ) ;
#34619=CARTESIAN_POINT ( 'NONE',  ( 35.81083249352388265, -277.0250047296078151, -260.6067658220363796 ) ) ;
#34620=CARTESIAN_POINT ( 'NONE',  ( -93.95033009541943159, -285.2746220978633573, -321.7037033135929960 ) ) ;
#34621=CARTESIAN_POINT ( 'NONE',  ( -18.64924441031904223, -281.6010559663841377, -341.3907197522622141 ) ) ;
#34622=CARTESIAN_POINT ( 'NONE',  ( -92.79221043608397679, -281.2570878009652233, -219.8612015835795717 ) ) ;
#34623=CARTESIAN_POINT ( 'NONE',  ( 38.49173738510147302, -275.5508976906021417, -256.9332699274085030 ) ) ;
#34624=CARTESIAN_POINT ( 'NONE',  ( 34.18346728356978304, -275.7488574620611530, -299.0206531995406749 ) ) ;
#34625=CARTESIAN_POINT ( 'NONE',  ( -85.38926932990192142, -297.6419874583990008, -327.2860134175114695 ) ) ;
#34628=CARTESIAN_POINT ( 'NONE',  ( -71.53807847860753100, -293.6386390701184155, -337.9696469675988055 ) ) ;
#34629=CARTESIAN_POINT ( 'NONE',  ( -7.488238461637044985, -276.1574788842698354, -337.0451435686070454 ) ) ;
#34630=CARTESIAN_POINT ( 'NONE',  ( 37.39547355830849540, -295.2665764641240571, -285.7579561074740013 ) ) ;
#34631=CARTESIAN_POINT ( 'NONE',  ( 37.39990805948450259, -294.9689610467435159, -287.2043182988343801 ) ) ;
#34632=CARTESIAN_POINT ( 'NONE',  ( -91.15187720228725254, -293.2853276991290841, -218.3563752242979206 ) ) ;
#34633=CARTESIAN_POINT ( 'NONE',  ( -111.9855820056045843, -276.6204681974154482, -265.0395277642510337 ) ) ;
#34634=CARTESIAN_POINT ( 'NONE',  ( -109.5633322116164692, -280.2382647869965240, -288.4510574660374118 ) ) ;
#34636=CARTESIAN_POINT ( 'NONE',  ( -95.07457378143783444, -293.9795390896061349, -317.3729614486250625 ) ) ;
#34637=CARTESIAN_POINT ( 'NONE',  ( -21.95334435352920366, -284.7174162525229235, -344.5467229499233781 ) ) ;
#34638=CARTESIAN_POINT ( 'NONE',  ( -30.48875328129863860, -285.0610285355732003, -197.3220008573639461 ) ) ;
#34639=CARTESIAN_POINT ( 'NONE',  ( -101.9332918901048117, -256.7340164629418382, -326.1142880538245095 ) ) ;
#34641=CARTESIAN_POINT ( 'NONE',  ( -89.67504842947793975, -284.9557429666089092, -219.3640283090289245 ) ) ;
#34643=CARTESIAN_POINT ( 'NONE',  ( 36.18627904402518425, -282.9084659525177585, -292.3413712554696531 ) ) ;
#34644=CARTESIAN_POINT ( 'NONE',  ( -110.5420146832385768, -283.6341187876053027, -247.6056614346497895 ) ) ;
#34645=CARTESIAN_POINT ( 'NONE',  ( -71.14182444028119789, -280.5581162100088477, -201.4381768772905446 ) ) ;
#34646=CARTESIAN_POINT ( 'NONE',  ( -96.50444023453960085, -279.4194594291496401, -318.5736677799964127 ) ) ;
#34647=CARTESIAN_POINT ( 'NONE',  ( -74.96531251642167604, -280.2159816878609604, -203.2956531177505610 ) ) ;
#34648=CARTESIAN_POINT ( 'NONE',  ( -6.998514795304330072, -274.1237833571632905, -333.4427485647536855 ) ) ;
#34649=CARTESIAN_POINT ( 'NONE',  ( 181.0651834200913015, 253.6962031844424246, -166.7746545555078512 ) ) ;
#34650=CARTESIAN_POINT ( 'NONE',  ( -82.18959793761349886, -275.4394140274640677, -210.3903658329570305 ) ) ;
#34651=CARTESIAN_POINT ( 'NONE',  ( 167.2772850727250784, 232.7340772729295963, -192.4600619714121592 ) ) ;
#34652=CARTESIAN_POINT ( 'NONE',  ( -79.97407639820484349, -277.4922446216823460, -209.0885523938139841 ) ) ;
#34653=CARTESIAN_POINT ( 'NONE',  ( 36.48095213073637666, -295.5411406815074997, -288.4209080095041600 ) ) ;
#34654=CARTESIAN_POINT ( 'NONE',  ( 29.95282405094631173, -292.5163581805219906, -241.6774244366818607 ) ) ;
#34655=CARTESIAN_POINT ( 'NONE',  ( -54.49400215255699464, -288.7743486719640487, -345.4179565856551335 ) ) ;
#34657=CARTESIAN_POINT ( 'NONE',  ( 26.01297138460396141, -292.6940688904533090, -313.0787009003353205 ) ) ;
#34658=CARTESIAN_POINT ( 'NONE',  ( -60.20736029322054605, -284.1505867716117564, -200.1927347946018756 ) ) ;
#34659=CARTESIAN_POINT ( 'NONE',  ( -17.11848132108027087, -294.1762869335290134, -198.8801473249683909 ) ) ;
#34660=CARTESIAN_POINT ( 'NONE',  ( -52.21008618926200029, -284.3381937310760463, -198.1832900402271207 ) ) ;
#34661=CARTESIAN_POINT ( 'NONE',  ( -101.4295112317074796, -286.3574518255425119, -234.2846269847509006 ) ) ;
#34663=CARTESIAN_POINT ( 'NONE',  ( -25.07089793714612824, -293.1462320493814673, -194.5834984239086509 ) ) ;
#34664=CARTESIAN_POINT ( 'NONE',  ( 34.76530516317772879, -282.1996563480080908, -282.1326187223264697 ) ) ;
#34665=CARTESIAN_POINT ( 'NONE',  ( 37.04008665724141736, -292.1168062012749829, -252.0483215077572368 ) ) ;
#34666=CARTESIAN_POINT ( 'NONE',  ( 18.53442655028765884, -289.0767740728888953, -323.1059498418403564 ) ) ;
#34667=CARTESIAN_POINT ( 'NONE',  ( -108.7390208684525703, -290.6803569414378217, -299.0307795463495495 ) ) ;
#34668=CARTESIAN_POINT ( 'NONE',  ( 35.12447126759131777, -287.8350800243681533, -279.1732691247583489 ) ) ;
#34671=CARTESIAN_POINT ( 'NONE',  ( -93.29060163430781927, -295.9536642686580308, -218.1013100128574820 ) ) ;
#34672=CARTESIAN_POINT ( 'NONE',  ( 29.19144475328732469, -280.1978750727375882, -239.6331852562164215 ) ) ;
#34674=CARTESIAN_POINT ( 'NONE',  ( -36.93375766454642672, -273.5648192455288381, -193.4106959168321964 ) ) ;
#34676=CARTESIAN_POINT ( 'NONE',  ( -61.25629503999773107, -293.8481334486833703, -340.1202990492721483 ) ) ;
#34677=CARTESIAN_POINT ( 'NONE',  ( 23.30892874303929219, -277.8967839646896323, -312.8693635667304989 ) ) ;
#34678=CARTESIAN_POINT ( 'NONE',  ( -109.1285212950539005, -270.9395726783268969, -251.2560937762742697 ) ) ;
#34679=CARTESIAN_POINT ( 'NONE',  ( -92.47887531243631543, -297.0693714036058282, -318.8071954112993467 ) ) ;
#34680=CARTESIAN_POINT ( 'NONE',  ( -104.2129662079976811, -297.2273845813862181, -300.5261238910584893 ) ) ;
#34682=CARTESIAN_POINT ( 'NONE',  ( -96.77057272029354351, -297.5062889878216765, -318.0750478232178580 ) ) ;
#34683=CARTESIAN_POINT ( 'NONE',  ( -107.6232271891730363, -270.9257671216616359, -243.0346446930340676 ) ) ;
#34684=CARTESIAN_POINT ( 'NONE',  ( -30.80610952973618311, -292.7883631844863999, -197.5519240320552683 ) ) ;
#34685=CARTESIAN_POINT ( 'NONE',  ( -97.69260231538486039, -273.9924029724693924, -222.8013931459084915 ) ) ;
#34686=CARTESIAN_POINT ( 'NONE',  ( -109.7619928982494883, -288.9559160894338561, -283.4254248234242368 ) ) ;
#34687=CARTESIAN_POINT ( 'NONE',  ( -54.69844564832022371, -275.8292287696853577, -197.3971266540792726 ) ) ;
#34688=CARTESIAN_POINT ( 'NONE',  ( -71.38122067187319431, -274.1069944372093232, -201.3622923063555277 ) ) ;
#34689=CARTESIAN_POINT ( 'NONE',  ( -110.2336450172874152, -296.9426953731224330, -266.0192454640999244 ) ) ;
#34690=CARTESIAN_POINT ( 'NONE',  ( -36.79046225364149336, -282.0389369794589811, -194.9951635931056444 ) ) ;
#34691=CARTESIAN_POINT ( 'NONE',  ( 24.20505700632235602, -279.6291621945156862, -224.9156015909709083 ) ) ;
#34692=CARTESIAN_POINT ( 'NONE',  ( -1.522573876527668402, -275.9384868606900341, -338.4074476517554331 ) ) ;
#34693=CARTESIAN_POINT ( 'NONE',  ( 18.58697806780103789, -279.2397000394237807, -218.6076314252914017 ) ) ;
#34694=CARTESIAN_POINT ( 'NONE',  ( 21.94090743705303836, -280.1846917446368934, -316.5944711029593464 ) ) ;
#34696=CARTESIAN_POINT ( 'NONE',  ( 9.876952651512992176, -273.2917661412396910, -213.8517153453059052 ) ) ;
#34697=CARTESIAN_POINT ( 'NONE',  ( -109.1561632495989329, -280.2731344996082612, -292.0311965347975729 ) ) ;
#34699=CARTESIAN_POINT ( 'NONE',  ( 29.69732919578551034, -297.1203304518544428, -194.3941983128116533 ) ) ;
#34700=CARTESIAN_POINT ( 'NONE',  ( 31.82488681210629622, -291.1828619517745551, -240.4547632895808817 ) ) ;
#34701=CARTESIAN_POINT ( 'NONE',  ( -79.59441708530674475, -291.4985942665006178, -205.9257428914671948 ) ) ;
#34703=CARTESIAN_POINT ( 'NONE',  ( -7.283849949174745930, -278.6590430220001053, -339.2702770704161139 ) ) ;
#34704=CARTESIAN_POINT ( 'NONE',  ( 6.362314196337084837, -272.6451177063137266, -209.3464440268392934 ) ) ;
#34706=CARTESIAN_POINT ( 'NONE',  ( -52.60242045280703849, -285.1661898677455724, -344.4174561643111474 ) ) ;
#34707=CARTESIAN_POINT ( 'NONE',  ( -82.94747669176435068, -281.6754900528038661, -329.9665625475703337 ) ) ;
#34709=CARTESIAN_POINT ( 'NONE',  ( -58.53749177896287392, -294.1273222991206353, -340.6310896649588926 ) ) ;
#34710=CARTESIAN_POINT ( 'NONE',  ( 35.49149907240992263, -285.8788575851584710, -284.7860628873933706 ) ) ;
#34712=CARTESIAN_POINT ( 'NONE',  ( -35.62981809008638834, -293.0305454668886114, -345.3544216147785164 ) ) ;
#34713=CARTESIAN_POINT ( 'NONE',  ( -111.2087277765731415, -282.7897069738754112, -289.5537661668501528 ) ) ;
#34714=CARTESIAN_POINT ( 'NONE',  ( -77.27164962212818011, -281.1075071840116379, -208.2353873607800097 ) ) ;
#34715=CARTESIAN_POINT ( 'NONE',  ( -110.3026459722295414, -285.4617810264124387, -293.7433513925200259 ) ) ;
#34716=CARTESIAN_POINT ( 'NONE',  ( 22.58968403144471537, -280.4246721441599561, -317.0961951208058167 ) ) ;
#34717=CARTESIAN_POINT ( 'NONE',  ( 16.89061578888612303, -286.8522754880038974, -221.4767638214944441 ) ) ;
#34718=CARTESIAN_POINT ( 'NONE',  ( -110.8681274788516475, -279.9376550229663962, -273.4007555625579471 ) ) ;
#34719=CARTESIAN_POINT ( 'NONE',  ( -107.3846605697953152, -279.6341552884568955, -249.2285502331041300 ) ) ;
#34720=CARTESIAN_POINT ( 'NONE',  ( -54.61264991168798133, -287.8111650511149264, -197.0118092379581185 ) ) ;
#34721=VERTEX_POINT ( 'NONE', #31894 ) ;
#34722=CARTESIAN_POINT ( 'NONE',  ( -65.54002848208352816, -297.5269281134641233, -198.6532097947270472 ) ) ;
#34723=CARTESIAN_POINT ( 'NONE',  ( -110.7930293011079783, -292.3605303445295931, -283.6558179571153460 ) ) ;
#34724=CARTESIAN_POINT ( 'NONE',  ( 151.9709352735115147, -299.5541904835127980, -193.4639945212225882 ) ) ;
#34725=CARTESIAN_POINT ( 'NONE',  ( 13.84574458161073096, -296.9090924074130839, -334.4957818155094174 ) ) ;
#34727=CARTESIAN_POINT ( 'NONE',  ( 29.62870018981954701, -273.1017076632485328, -236.2291109395855813 ) ) ;
#34728=CARTESIAN_POINT ( 'NONE',  ( -64.00553827083086844, -293.7940943842461934, -341.7437499775447804 ) ) ;
#34729=CARTESIAN_POINT ( 'NONE',  ( -37.81663015600997824, -297.5536962934498320, -197.3011228871214939 ) ) ;
#34730=CARTESIAN_POINT ( 'NONE',  ( 24.83360661913408052, -289.6140798987131006, -309.9204276691947371 ) ) ;
#34731=CARTESIAN_POINT ( 'NONE',  ( 3.241139586490572100, -282.3653760001507180, -208.4045026555773177 ) ) ;
#34732=CARTESIAN_POINT ( 'NONE',  ( -65.21503782004542416, -290.8345052616252246, -341.5625315729826070 ) ) ;
#34733=CARTESIAN_POINT ( 'NONE',  ( -113.8964770739265759, -291.8562635233860760, -271.2399166129128503 ) ) ;
#34734=CARTESIAN_POINT ( 'NONE',  ( -63.27777232619048675, -287.7145853110660028, -199.9329974921880080 ) ) ;
#34735=CARTESIAN_POINT ( 'NONE',  ( -45.27548226331739301, -280.1211034760565894, -193.7179512911521613 ) ) ;
#34736=CARTESIAN_POINT ( 'NONE',  ( 30.91844896985933389, -292.0565619899851981, -302.8846438870362476 ) ) ;
#34737=CARTESIAN_POINT ( 'NONE',  ( 6.186003030231581157, -280.4586625390465997, -206.8446708034898336 ) ) ;
#34738=CARTESIAN_POINT ( 'NONE',  ( 31.30820270979395303, -277.0386460713366432, -241.9763546344181862 ) ) ;
#34739=CARTESIAN_POINT ( 'NONE',  ( -102.0455923789670294, -281.4805209788416960, -239.2376011013261916 ) ) ;
#34742=CARTESIAN_POINT ( 'NONE',  ( 27.83912614869473856, -280.6106913460508849, -237.2421286811087100 ) ) ;
#34743=CARTESIAN_POINT ( 'NONE',  ( -42.76267528196521539, -278.3242009645552457, -346.7719925168307782 ) ) ;
#34745=CARTESIAN_POINT ( 'NONE',  ( -110.0732731638158413, -274.0101703223464824, -259.4599821788766576 ) ) ;
#34746=CARTESIAN_POINT ( 'NONE',  ( -21.02226692331584346, -285.3153897219928012, -195.3511432314969909 ) ) ;
#34747=CARTESIAN_POINT ( 'NONE',  ( -95.93009435832956910, -292.9402799989143773, -225.1353059088673092 ) ) ;
#34748=CARTESIAN_POINT ( 'NONE',  ( -95.43118985042337954, -274.8242034420152322, -221.0251858657978232 ) ) ;
#34749=CARTESIAN_POINT ( 'NONE',  ( -113.0587449782604779, -274.0098918034981352, -259.0344129169586722 ) ) ;
#34751=CARTESIAN_POINT ( 'NONE',  ( 30.27722583338860574, -275.7555522813397602, -298.0034445799832952 ) ) ;
#34752=CARTESIAN_POINT ( 'NONE',  ( -101.7312792821809211, -298.0399770336214260, -308.5945826886912187 ) ) ;
#34753=CARTESIAN_POINT ( 'NONE',  ( -86.07449729940954342, -281.7294940858326413, -327.1514596211674188 ) ) ;
#34754=CARTESIAN_POINT ( 'NONE',  ( -73.42004688929604583, -291.2536529461331156, -202.3455080813807854 ) ) ;
#34755=CARTESIAN_POINT ( 'NONE',  ( 6.339335130137395247, -274.4762028274008117, -330.9543790818390789 ) ) ;
#34756=CARTESIAN_POINT ( 'NONE',  ( 32.14380682227470487, -289.5559589520439090, -301.6373827419291729 ) ) ;
#34757=CARTESIAN_POINT ( 'NONE',  ( -108.9676805778728408, -289.2665994215886940, -286.0382648058151176 ) ) ;
#34759=CARTESIAN_POINT ( 'NONE',  ( -113.4183534413896126, -289.2237107660537276, -262.6780196637561176 ) ) ;
#34760=CARTESIAN_POINT ( 'NONE',  ( -91.68605695289608093, -290.9168724163483262, -221.5696955242788704 ) ) ;
#34762=CARTESIAN_POINT ( 'NONE',  ( 26.87139715829713893, -288.0787222663853981, -228.4305724765549428 ) ) ;
#34763=CARTESIAN_POINT ( 'NONE',  ( -99.48795644756521028, -279.4150983156598613, -231.9249773438579609 ) ) ;
#34765=CARTESIAN_POINT ( 'NONE',  ( -99.76494437933996551, -294.8789718650247664, -315.0020282840965251 ) ) ;
#34766=CARTESIAN_POINT ( 'NONE',  ( -67.83329611510730217, -284.0933995540761430, -340.9555608303939493 ) ) ;
#34767=CARTESIAN_POINT ( 'NONE',  ( -54.96389174355455509, -286.1648190338543145, -195.4264620875560752 ) ) ;
#34768=CARTESIAN_POINT ( 'NONE',  ( 7.810364288832802870, -282.7494330902450201, -327.8136630376168910 ) ) ;
#34769=CARTESIAN_POINT ( 'NONE',  ( -22.11190715825497932, -108.2714217967105412, -362.7848814367727641 ) ) ;
#34770=CARTESIAN_POINT ( 'NONE',  ( 137.5487510745606983, 180.6726423773487227, -240.5649509146122398 ) ) ;
#34771=CARTESIAN_POINT ( 'NONE',  ( 166.3627146848736515, 230.6933907105903927, -190.1005024542335491 ) ) ;
#34772=CARTESIAN_POINT ( 'NONE',  ( 35.26502700774396715, -274.8729917950416848, -279.7571910365083454 ) ) ;
#34773=CARTESIAN_POINT ( 'NONE',  ( -31.30058955305620216, -273.0505344411276951, -197.2886374975107060 ) ) ;
#34774=CARTESIAN_POINT ( 'NONE',  ( -5.828644376177721576, -294.1564680192196874, -340.5498223488882559 ) ) ;
#34775=CARTESIAN_POINT ( 'NONE',  ( -104.6679026044236309, -261.1202776925566127, -315.8143883333635245 ) ) ;
#34776=CARTESIAN_POINT ( 'NONE',  ( 20.43675060126592413, -274.9192535372062594, -320.5302067277217475 ) ) ;
#34777=CARTESIAN_POINT ( 'NONE',  ( -66.07227665129953209, -299.5325181877643672, -201.9109941376503627 ) ) ;
#34778=CARTESIAN_POINT ( 'NONE',  ( -20.01237063769642077, -293.3596810881329020, -199.0771729337055262 ) ) ;
#34780=CARTESIAN_POINT ( 'NONE',  ( -110.1188164666183980, -297.1849533066197182, -294.7806091769484169 ) ) ;
#34781=CARTESIAN_POINT ( 'NONE',  ( 34.05480907052476169, -287.8400844654296975, -254.8521877769566686 ) ) ;
#34782=CARTESIAN_POINT ( 'NONE',  ( -112.9819640328105805, -297.5243853509301175, -256.8441176792582610 ) ) ;
#34783=CARTESIAN_POINT ( 'NONE',  ( -22.10359825035988024, -295.3543095286810853, -345.7754876624986196 ) ) ;
#34784=CARTESIAN_POINT ( 'NONE',  ( 33.64726771441192454, -293.4936948443024676, -253.2910701396889408 ) ) ;
#34786=CARTESIAN_POINT ( 'NONE',  ( 37.30119535383369112, -277.3216613804019062, -258.5410928806853690 ) ) ;
#34789=CARTESIAN_POINT ( 'NONE',  ( 12.95667890233088926, -280.2405265742137885, -212.1408468566241936 ) ) ;
#34790=CARTESIAN_POINT ( 'NONE',  ( -2.813278050477213910, -275.4617399140823295, -205.7763170040344676 ) ) ;
#34791=CARTESIAN_POINT ( 'NONE',  ( 37.72302324545031382, -277.1616743738731543, -258.4764993362041423 ) ) ;
#34792=CARTESIAN_POINT ( 'NONE',  ( -42.71460500694947626, -275.1397471290803196, -345.5245312669811710 ) ) ;
#34793=CARTESIAN_POINT ( 'NONE',  ( -57.94143701328127349, -298.4303232501237062, -200.2216604128813913 ) ) ;
#34794=CARTESIAN_POINT ( 'NONE',  ( -110.6881158728572956, -295.0408554218947756, -276.9343593594032882 ) ) ;
#34796=CARTESIAN_POINT ( 'NONE',  ( -112.6585964759462541, -279.2419554157448260, -254.5847601917703287 ) ) ;
#34797=CARTESIAN_POINT ( 'NONE',  ( 5.398504748897619443, -276.6224295686203618, -329.6035624467439220 ) ) ;
#34798=CARTESIAN_POINT ( 'NONE',  ( 25.15202228337788526, -285.6489470938124668, -226.2042640086056906 ) ) ;
#34799=CARTESIAN_POINT ( 'NONE',  ( 6.623143572226626752, -300.6014512949777782, -195.1794950382704030 ) ) ;
#34801=CARTESIAN_POINT ( 'NONE',  ( 16.12199045057448288, -287.4667401769644357, -320.3775553551095072 ) ) ;
#34802=ADVANCED_FACE ( 'NONE', ( #29693 ), #15621, .T. ) ;
#34803=CARTESIAN_POINT ( 'NONE',  ( -57.36613410449184869, -278.0300052831409516, -199.1080755551348886 ) ) ;
#34804=CARTESIAN_POINT ( 'NONE',  ( -109.1780148339836387, -277.3364987196846414, -254.3373215321235818 ) ) ;
#34805=CARTESIAN_POINT ( 'NONE',  ( -29.31317892787824420, -281.0296350217703889, -344.4184079500287794 ) ) ;
#34807=CARTESIAN_POINT ( 'NONE',  ( -73.18439904005735741, -287.5771708395021165, -204.4658021102520422 ) ) ;
#34808=CARTESIAN_POINT ( 'NONE',  ( -35.09016331039060788, -278.2283300456271604, -343.7236498893889802 ) ) ;
#34810=CARTESIAN_POINT ( 'NONE',  ( -97.61296734770746752, -293.1617239487760571, -225.7035667479326548 ) ) ;
#34811=CARTESIAN_POINT ( 'NONE',  ( -90.63453748185219183, -276.0343375893257871, -324.5998270100259901 ) ) ;
#34812=CARTESIAN_POINT ( 'NONE',  ( -1.680142477784674737, -275.1894711722507054, -206.5334170151342619 ) ) ;
#34813=CARTESIAN_POINT ( 'NONE',  ( 34.72836271182631407, -283.8288064465004936, -291.8930104289210590 ) ) ;
#34815=CARTESIAN_POINT ( 'NONE',  ( 24.68391636086507646, -290.0544256198056701, -313.6034794155489180 ) ) ;
#34816=CARTESIAN_POINT ( 'NONE',  ( -105.4139788496644030, -294.1370311131459516, -301.9660448810851108 ) ) ;
#34818=CARTESIAN_POINT ( 'NONE',  ( -35.36035753594892839, -272.7623271764321089, -196.8820886809818944 ) ) ;
#34819=CARTESIAN_POINT ( 'NONE',  ( 36.52690191429072541, -291.5896792283005539, -262.4941703303803138 ) ) ;
#34820=CARTESIAN_POINT ( 'NONE',  ( 207.9737475149031525, 296.4638663539913637, -68.98948423471202318 ) ) ;
#34822=CARTESIAN_POINT ( 'NONE',  ( -97.78706769693164347, -289.6594086705076165, -223.7667576904704276 ) ) ;
#34823=CARTESIAN_POINT ( 'NONE',  ( 37.03631310405469890, -285.5941160179363578, -254.7453713818323990 ) ) ;
#34824=CARTESIAN_POINT ( 'NONE',  ( -106.1220527560646616, -286.3239754578983707, -244.1955297318808675 ) ) ;
#34826=CARTESIAN_POINT ( 'NONE',  ( -104.7503082324676029, -285.7373738153922886, -241.7935368588081246 ) ) ;
#34827=CARTESIAN_POINT ( 'NONE',  ( -112.4704175978014149, -292.4492774925226968, -276.8378661692688638 ) ) ;
#34829=CARTESIAN_POINT ( 'NONE',  ( 35.83789687934412882, -273.8719728185081976, -289.1776209214245910 ) ) ;
#34830=CARTESIAN_POINT ( 'NONE',  ( 27.63326298442649431, -276.4277087081979971, -311.7397266418570325 ) ) ;
#34831=CARTESIAN_POINT ( 'NONE',  ( -94.55426840664475208, -289.3114171849274499, -220.9851317030108646 ) ) ;
#34832=CARTESIAN_POINT ( 'NONE',  ( 1.047033484055708508, -276.5548809108971682, -337.1696683886106030 ) ) ;
#34833=CARTESIAN_POINT ( 'NONE',  ( -96.05184441720986399, -297.8962955894935476, -316.4584689309289729 ) ) ;
#34836=CARTESIAN_POINT ( 'NONE',  ( -100.8355526829287214, -282.7324501029693806, -307.3715781910439091 ) ) ;
#34837=CARTESIAN_POINT ( 'NONE',  ( -25.68076379665600939, -278.2005651171000977, -196.2731755745033979 ) ) ;
#34839=CARTESIAN_POINT ( 'NONE',  ( 38.68802916633765676, -274.1140019187301959, -276.8563481443550813 ) ) ;
#34840=CARTESIAN_POINT ( 'NONE',  ( -96.97364705169449905, -277.3108886947960059, -312.6667065204230198 ) ) ;
#34841=CARTESIAN_POINT ( 'NONE',  ( 32.20071665298686270, -295.3954400826411870, -294.8976309867817918 ) ) ;
#34842=CARTESIAN_POINT ( 'NONE',  ( 38.87717864663719070, -280.3599579046581880, -261.3997930701264636 ) ) ;
#34843=CARTESIAN_POINT ( 'NONE',  ( -47.81487395849057265, -296.1297233655395189, -342.8951192446049276 ) ) ;
#34844=CARTESIAN_POINT ( 'NONE',  ( -34.85379651485801134, -296.3366775125805361, -346.8275067401354477 ) ) ;
#34845=CARTESIAN_POINT ( 'NONE',  ( -110.3628441122352086, -272.2189246215068579, -270.3568844605550225 ) ) ;
#34846=CARTESIAN_POINT ( 'NONE',  ( -47.28413701110132195, -293.9259653710377052, -196.0230483558537458 ) ) ;
#34847=CARTESIAN_POINT ( 'NONE',  ( -109.9779594186021541, -285.0411874913648944, -244.8077651540625936 ) ) ;
#34848=CARTESIAN_POINT ( 'NONE',  ( -31.33399846250000564, -272.2668211581582796, -194.8218091159841663 ) ) ;
#34849=CARTESIAN_POINT ( 'NONE',  ( -32.30429976689524807, -285.9473153225691249, -193.5129037078436340 ) ) ;
#34850=CARTESIAN_POINT ( 'NONE',  ( -105.9638482691047727, -280.9179354070602130, -240.9868505978010091 ) ) ;
#34851=CARTESIAN_POINT ( 'NONE',  ( -39.97039889651348687, -285.0770602528756967, -197.1730151826463668 ) ) ;
#34852=CARTESIAN_POINT ( 'NONE',  ( -43.05599790272027150, -287.1241451349372369, -345.1431174888140845 ) ) ;
#34853=CARTESIAN_POINT ( 'NONE',  ( 202.9738562182569694, 291.4636489450776367, -54.00000000000002132 ) ) ;
#34854=CARTESIAN_POINT ( 'NONE',  ( -38.61970067576419297, -285.5433849438857123, -197.2982652854080925 ) ) ;
#34855=CARTESIAN_POINT ( 'NONE',  ( -63.81957747868795394, -284.3303814239517919, -342.4148633659583538 ) ) ;
#34856=CARTESIAN_POINT ( 'NONE',  ( -68.22307855902910489, -290.7151550034422485, -200.0676336702732385 ) ) ;
#34857=CARTESIAN_POINT ( 'NONE',  ( -112.0056208560555859, -279.9590775985041091, -285.6485065458944064 ) ) ;
#34858=CARTESIAN_POINT ( 'NONE',  ( -105.8960037863007528, -279.4266203238732373, -304.4450316289065199 ) ) ;
#34859=CARTESIAN_POINT ( 'NONE',  ( 30.02230883784898552, -281.0081782901216343, -242.2347904490163444 ) ) ;
#34860=CARTESIAN_POINT ( 'NONE',  ( 28.37707973213417390, -277.0705438251273449, -234.1137325286281623 ) ) ;
#34861=CARTESIAN_POINT ( 'NONE',  ( -36.27444894065352798, -295.0391552500411763, -347.3668250999490397 ) ) ;
#34862=CARTESIAN_POINT ( 'NONE',  ( -90.98113109435963963, -289.3059168997201596, -218.4510202373755305 ) ) ;
#34863=CARTESIAN_POINT ( 'NONE',  ( -106.9961918954946754, -295.7764794663020780, -247.3425047631344569 ) ) ;
#34864=VERTEX_POINT ( 'NONE', #60327 ) ;
#34866=CARTESIAN_POINT ( 'NONE',  ( 30.63930732748062269, -283.8742929518865026, -300.8175764710408089 ) ) ;
#34867=CARTESIAN_POINT ( 'NONE',  ( -100.1868323992704291, -295.7069111884517270, -307.6437073652548406 ) ) ;
#34868=CARTESIAN_POINT ( 'NONE',  ( 38.30367642553348873, -294.7912890927890999, -283.0609753807915467 ) ) ;
#34869=CARTESIAN_POINT ( 'NONE',  ( -5.981698428774349985, -283.2801980118110805, -336.4085383071718525 ) ) ;
#34870=CARTESIAN_POINT ( 'NONE',  ( 38.49703156754828370, -274.4607172271563513, -258.3890429680355965 ) ) ;
#34871=CARTESIAN_POINT ( 'NONE',  ( -53.37617266193706200, -292.5032411105555639, -195.0989225402719001 ) ) ;
#34872=CARTESIAN_POINT ( 'NONE',  ( -82.52003460816783331, -283.5824377822683005, -209.4744674429073541 ) ) ;
#34874=CARTESIAN_POINT ( 'NONE',  ( -113.1519346539427744, -291.0525925022996603, -256.9987591825890263 ) ) ;
#34875=CARTESIAN_POINT ( 'NONE',  ( -15.84137413978352704, -289.0996573495766029, -340.1980800740345217 ) ) ;
#34877=CARTESIAN_POINT ( 'NONE',  ( 151.9709352735115147, -299.5541904835127980, -197.7582414438974183 ) ) ;
#34878=CARTESIAN_POINT ( 'NONE',  ( -93.57506545626765160, -238.8899425540025732, -338.5510770644321497 ) ) ;
#34880=CARTESIAN_POINT ( 'NONE',  ( -71.41164631641019866, -285.0140381376205596, -338.6395664266647145 ) ) ;
#34881=CARTESIAN_POINT ( 'NONE',  ( -106.6379572354042296, -288.4809262143061801, -236.9535640164627353 ) ) ;
#34883=CARTESIAN_POINT ( 'NONE',  ( -76.97747113672873809, -278.4281391505144256, -208.6302636669330468 ) ) ;
#34884=CARTESIAN_POINT ( 'NONE',  ( -22.94701782041445526, -276.5396826626063671, -346.0362993238227887 ) ) ;
#34885=CARTESIAN_POINT ( 'NONE',  ( -86.28554348697379339, -279.7328562816900330, -327.0382947923185384 ) ) ;
#34886=CARTESIAN_POINT ( 'NONE',  ( 204.3871895515903248, 292.5236489450776958, -53.99999999999455014 ) ) ;
#34887=CARTESIAN_POINT ( 'NONE',  ( 36.76427342440241119, -279.8920491580465182, -251.7355715855615301 ) ) ;
#34888=CARTESIAN_POINT ( 'NONE',  ( -98.69378116030685533, -283.1518735600507739, -227.8206685669494789 ) ) ;
#34889=CARTESIAN_POINT ( 'NONE',  ( -112.1455606784105186, -298.4815393233037639, -257.0061016257323558 ) ) ;
#34890=CARTESIAN_POINT ( 'NONE',  ( 21.37966315882518842, -294.6534933974772343, -313.8328321831493213 ) ) ;
#34892=CARTESIAN_POINT ( 'NONE',  ( -107.4274312687419979, -288.9437451264233800, -292.6481920682344935 ) ) ;
#34893=CARTESIAN_POINT ( 'NONE',  ( -29.85706811716175579, -274.7959605023299332, -193.8281638375711395 ) ) ;
#34894=CARTESIAN_POINT ( 'NONE',  ( -33.81424395968752350, -298.2642020799203237, -197.3610147765085685 ) ) ;
#34899=CARTESIAN_POINT ( 'NONE',  ( -2.268733174508112516, -283.6561238650434689, -334.7502549594791503 ) ) ;
#34900=CARTESIAN_POINT ( 'NONE',  ( -72.06402642006176507, -281.3595705509151230, -202.7572053406856583 ) ) ;
#34901=CARTESIAN_POINT ( 'NONE',  ( -110.5545463210118555, -283.5678223541961529, -273.6367442581140494 ) ) ;
#34902=CARTESIAN_POINT ( 'NONE',  ( 36.58003424204504483, -283.3171595060405252, -263.0057923563188069 ) ) ;
#34903=CARTESIAN_POINT ( 'NONE',  ( 35.31244880180084067, -273.8698938981283391, -257.9538829502668591 ) ) ;
#34906=CARTESIAN_POINT ( 'NONE',  ( -86.98306216611699426, -278.5254089173731131, -329.0813367292180942 ) ) ;
#34910=CARTESIAN_POINT ( 'NONE',  ( -109.3616792153565882, -286.8185728203726512, -248.0148332090969348 ) ) ;
#34911=CARTESIAN_POINT ( 'NONE',  ( 26.38021410812946854, -292.2571471555543781, -234.3115893274394921 ) ) ;
#34912=CARTESIAN_POINT ( 'NONE',  ( -23.33865316137603330, -288.2263450277679908, -346.0275100325083031 ) ) ;
#34913=CARTESIAN_POINT ( 'NONE',  ( -109.3461984836874592, -283.0155039983598044, -253.1798373346379947 ) ) ;
#34914=CARTESIAN_POINT ( 'NONE',  ( -67.77493950686475443, -284.2194285512869669, -203.3596787471119001 ) ) ;
#34915=CARTESIAN_POINT ( 'NONE',  ( 22.77181050501753745, -286.3873776472089503, -313.5391199532005544 ) ) ;
#34916=CARTESIAN_POINT ( 'NONE',  ( 35.09791540649243302, -282.9122698011261150, -282.1777421405919313 ) ) ;
#34917=CARTESIAN_POINT ( 'NONE',  ( -3.438236613605195835, -272.4995135901275489, -203.4472000419003734 ) ) ;
#34918=CARTESIAN_POINT ( 'NONE',  ( -101.8304722108719176, -283.4891640215544157, -229.7700020852078922 ) ) ;
#34919=CARTESIAN_POINT ( 'NONE',  ( -64.83325620725437943, -299.6934189815007130, -200.5258398211536530 ) ) ;
#34920=CARTESIAN_POINT ( 'NONE',  ( -102.4396543298571913, -283.0536750585918071, -232.6772915953402503 ) ) ;
#34921=CARTESIAN_POINT ( 'NONE',  ( 35.26444115834450344, -282.3625003152594672, -260.4055710915121722 ) ) ;
#34922=CARTESIAN_POINT ( 'NONE',  ( 37.15481515015898850, -289.4240087408247177, -260.3462471551367798 ) ) ;
#34925=CARTESIAN_POINT ( 'NONE',  ( 24.54947000265249812, -296.0566078392772624, -313.7288034762532334 ) ) ;
#34926=CARTESIAN_POINT ( 'NONE',  ( -110.8423043290764838, -276.7444154510166072, -255.3748753844917587 ) ) ;
#34927=CARTESIAN_POINT ( 'NONE',  ( -107.5879083662718045, -289.3496447778621814, -301.6308894866839978 ) ) ;
#34928=CARTESIAN_POINT ( 'NONE',  ( -37.01222086387058852, -293.4477971240663123, -344.1729452613232070 ) ) ;
#34929=CARTESIAN_POINT ( 'NONE',  ( -95.16856964639428895, -277.8724360898360146, -224.9834368949919110 ) ) ;
#34930=CARTESIAN_POINT ( 'NONE',  ( -110.5412695400865033, -270.8106245447466449, -256.5530495532083819 ) ) ;
#34931=CARTESIAN_POINT ( 'NONE',  ( -104.0106643317493536, -292.2819877342362815, -239.4339019974963492 ) ) ;
#34932=CARTESIAN_POINT ( 'NONE',  ( -110.4542110544635705, -292.8376638359844719, -287.0812184334320705 ) ) ;
#34933=CARTESIAN_POINT ( 'NONE',  ( -108.2371887829772277, -295.3949219677122073, -241.9962210214575293 ) ) ;
#34934=CARTESIAN_POINT ( 'NONE',  ( -66.62795018090679378, -291.0422854302788096, -338.1560749579778076 ) ) ;
#34935=CARTESIAN_POINT ( 'NONE',  ( 23.18188603638981959, -291.1714037175487988, -224.3954982932913538 ) ) ;
#34936=CARTESIAN_POINT ( 'NONE',  ( -110.8352560569916818, -292.0382130484377967, -265.7163704602006646 ) ) ;
#34939=CARTESIAN_POINT ( 'NONE',  ( -79.63236048067405193, -292.2673751024350963, -210.5989172900428059 ) ) ;
#34941=CARTESIAN_POINT ( 'NONE',  ( -111.5336027501511893, -291.5167690566263445, -289.4810705395530590 ) ) ;
#34942=CARTESIAN_POINT ( 'NONE',  ( 35.94274053605528962, -279.7971243591792359, -287.9602393055343441 ) ) ;
#34943=CARTESIAN_POINT ( 'NONE',  ( 35.29532958035327539, -293.4497953869568505, -262.6019146164438780 ) ) ;
#34944=CARTESIAN_POINT ( 'NONE',  ( -8.861111436926220719, -280.4146078811587586, -198.8219254528337103 ) ) ;
#34946=CARTESIAN_POINT ( 'NONE',  ( 37.84395955264712796, -281.4262776350673221, -286.9404779621531816 ) ) ;
#34947=CARTESIAN_POINT ( 'NONE',  ( -10.07936173475944486, -286.6953941858417920, -340.1073845675351208 ) ) ;
#34948=CARTESIAN_POINT ( 'NONE',  ( 35.55156021711645309, -279.5085891333641825, -256.2427748035584614 ) ) ;
#34949=CARTESIAN_POINT ( 'NONE',  ( -54.48213658813285321, -283.8317529041719922, -197.3460093845242511 ) ) ;
#34951=CARTESIAN_POINT ( 'NONE',  ( 30.11800450644896898, -279.5660576432097741, -234.5847649902923706 ) ) ;
#34952=CARTESIAN_POINT ( 'NONE',  ( 16.09370281646036105, -285.7092527622109515, -215.3506624183742701 ) ) ;
#34953=CARTESIAN_POINT ( 'NONE',  ( 35.17922642174686132, -276.2278375210231047, -260.7010486603462596 ) ) ;
#34955=CARTESIAN_POINT ( 'NONE',  ( 23.99493740568049560, -294.5884971453511412, -229.3214138984063197 ) ) ;
#34956=CARTESIAN_POINT ( 'NONE',  ( 4.525022822553224522, -276.0300438007862454, -206.3782131517272660 ) ) ;
#34957=CARTESIAN_POINT ( 'NONE',  ( -66.81508685788679713, -277.1160456262686012, -337.1698521534723341 ) ) ;
#34958=CARTESIAN_POINT ( 'NONE',  ( -113.6664331571216877, -290.8509697137596959, -259.7954640900600225 ) ) ;
#34959=CARTESIAN_POINT ( 'NONE',  ( -100.2343974470069554, -282.0692527251739534, -312.3337110748246914 ) ) ;
#34960=CARTESIAN_POINT ( 'NONE',  ( -17.35691110858699560, -291.3750699415616623, -199.8525752498121051 ) ) ;
#34961=CARTESIAN_POINT ( 'NONE',  ( -52.89989665120770468, -293.2512535387423895, -343.7827918696546590 ) ) ;
#34964=CARTESIAN_POINT ( 'NONE',  ( 31.86134602843300456, -292.7468925525474219, -246.7744006299952559 ) ) ;
#34966=CARTESIAN_POINT ( 'NONE',  ( -53.35057174420112602, -280.7666405000205145, -340.3538533559490702 ) ) ;
#34967=CARTESIAN_POINT ( 'NONE',  ( -112.3777110944119357, -295.4076895070623436, -286.5604164944611512 ) ) ;
#34968=CARTESIAN_POINT ( 'NONE',  ( -96.77861483662742614, -285.2168214329187208, -318.5538026829544833 ) ) ;
#34969=CARTESIAN_POINT ( 'NONE',  ( 31.84127136285350801, -287.0759960627252099, -247.0648423105714073 ) ) ;
#34970=CARTESIAN_POINT ( 'NONE',  ( 23.04500141755317344, -277.6568034566590768, -312.6880038354847215 ) ) ;
#34971=CARTESIAN_POINT ( 'NONE',  ( -105.2036517932926785, -294.9837849558356311, -239.1465715141204669 ) ) ;
#34972=CARTESIAN_POINT ( 'NONE',  ( -98.00120783608370800, -297.7290415774002668, -312.7686425383072333 ) ) ;
#34973=CARTESIAN_POINT ( 'NONE',  ( 27.10811842817485839, -274.8251463079134282, -305.5864290773352536 ) ) ;
#34976=CARTESIAN_POINT ( 'NONE',  ( -101.5297151710278030, -296.7782490845821144, -227.8442588243519253 ) ) ;
#34977=CARTESIAN_POINT ( 'NONE',  ( -26.23637979520668750, -290.8300022091412984, -344.0201461410976549 ) ) ;
#34978=CARTESIAN_POINT ( 'NONE',  ( 202.7107630375198255, 295.9505694800565720, -54.00000000005820056 ) ) ;
#34979=CARTESIAN_POINT ( 'NONE',  ( 22.83852374697876897, -288.7809803426674762, -311.8829848586217395 ) ) ;
#34981=CARTESIAN_POINT ( 'NONE',  ( -5.032081409135720662, -279.5259625961167558, -200.7270117400689458 ) ) ;
#34982=CARTESIAN_POINT ( 'NONE',  ( -99.84354733968551443, -297.7979727864587289, -225.5634407895096558 ) ) ;
#34983=CARTESIAN_POINT ( 'NONE',  ( -108.3084050590193925, -289.0345037291086783, -243.6781269526779852 ) ) ;
#34984=CARTESIAN_POINT ( 'NONE',  ( -113.9217547311807124, -296.7875359790674565, -278.1866868729893554 ) ) ;
#34985=CARTESIAN_POINT ( 'NONE',  ( 29.87354671900513381, -293.5008940983319121, -241.6976179229490072 ) ) ;
#34988=CARTESIAN_POINT ( 'NONE',  ( -12.43160647034326338, -290.2542039735134267, -342.5427356789984970 ) ) ;
#34989=CARTESIAN_POINT ( 'NONE',  ( 40.64545035920995986, -283.8376638359844719, -252.5284128619064461 ) ) ;
#34991=CARTESIAN_POINT ( 'NONE',  ( 39.31076506226148126, -280.8238365130334842, -264.2200784456269957 ) ) ;
#34992=CARTESIAN_POINT ( 'NONE',  ( 15.23032876038422145, -284.3084113701843307, -323.6901844011642879 ) ) ;
#34994=CARTESIAN_POINT ( 'NONE',  ( 36.80945472854773470, -285.8943480812585562, -251.9162669860722303 ) ) ;
#34995=CARTESIAN_POINT ( 'NONE',  ( -81.27673970728709207, -287.7340103903598560, -330.5170934129919829 ) ) ;
#34996=CARTESIAN_POINT ( 'NONE',  ( 38.31928946176864770, -277.3507204399658121, -265.4951130508255801 ) ) ;
#34998=CARTESIAN_POINT ( 'NONE',  ( -102.1558831289512312, -279.0102546039531717, -236.6635809296179502 ) ) ;
#34999=CARTESIAN_POINT ( 'NONE',  ( 33.86155837230335663, -280.6826821099535891, -253.8085155434326907 ) ) ;
#35000=CARTESIAN_POINT ( 'NONE',  ( 28.83617688386293665, -277.1382940207387264, -309.1165189390781620 ) ) ;
#35001=CARTESIAN_POINT ( 'NONE',  ( -69.78019392368931051, -278.4294387159051780, -200.9511783809121255 ) ) ;
#35002=CARTESIAN_POINT ( 'NONE',  ( -84.79127711417702074, -218.1117258539772763, -350.1014080083962767 ) ) ;
#35003=CARTESIAN_POINT ( 'NONE',  ( -114.1064060109667508, -273.4932526720010628, -270.3730758795568363 ) ) ;
#35004=CARTESIAN_POINT ( 'NONE',  ( -36.56645602178579679, -299.4869440493469028, -193.9501587921773762 ) ) ;
#35005=CARTESIAN_POINT ( 'NONE',  ( -69.85430415644619018, -291.9805209788416391, -337.9475929042657754 ) ) ;
#35008=CARTESIAN_POINT ( 'NONE',  ( 23.77476431663124146, -289.1914790262187012, -310.8686655463697548 ) ) ;
#35009=CARTESIAN_POINT ( 'NONE',  ( -2.705076435574930827, -288.2638079838026215, -202.7131500892564588 ) ) ;
#35010=CARTESIAN_POINT ( 'NONE',  ( 32.77008559830159840, -286.6267683397261976, -249.6232196799394956 ) ) ;
#35011=CARTESIAN_POINT ( 'NONE',  ( -63.89666356167938943, -282.8970134293133469, -342.5716492105353836 ) ) ;
#35012=CARTESIAN_POINT ( 'NONE',  ( -71.29175051220498460, -277.9960376746051338, -204.8195209370862528 ) ) ;
#35013=CARTESIAN_POINT ( 'NONE',  ( 27.43379844523405353, -288.9235344496933635, -233.9930692874836211 ) ) ;
#35014=CARTESIAN_POINT ( 'NONE',  ( 0.7749871145252934523, -279.0499621532649144, -207.2320315072333017 ) ) ;
#35015=CARTESIAN_POINT ( 'NONE',  ( -95.65415360224463370, -279.2421997414294879, -315.0925526705166249 ) ) ;
#35016=CARTESIAN_POINT ( 'NONE',  ( 21.52704858610170646, -275.4387243879731386, -227.0892002225640454 ) ) ;
#35017=CARTESIAN_POINT ( 'NONE',  ( 35.56510900238991724, -286.6442381895781750, -293.8686891211037846 ) ) ;
#35019=CARTESIAN_POINT ( 'NONE',  ( 9.119308708470402536, -283.2351032242546580, -331.5618816860834954 ) ) ;
#35020=CARTESIAN_POINT ( 'NONE',  ( -88.27609999514243100, -284.2352236190148460, -328.0969160817451211 ) ) ;
#35021=CARTESIAN_POINT ( 'NONE',  ( -21.38614744700854331, -283.0086018331040805, -341.6480968521278783 ) ) ;
#35025=CARTESIAN_POINT ( 'NONE',  ( -15.28876965590376180, -290.6301743983809729, -342.9002802508434229 ) ) ;
#35026=CARTESIAN_POINT ( 'NONE',  ( -66.80992407303810410, -290.3588327283977151, -199.7571375642989153 ) ) ;
#35027=CARTESIAN_POINT ( 'NONE',  ( -47.28459635517239690, -297.1198846279776262, -197.8271035934619135 ) ) ;
#35028=CARTESIAN_POINT ( 'NONE',  ( 39.34004276821458035, -292.8285587788984685, -264.5971703139227884 ) ) ;
#35029=CARTESIAN_POINT ( 'NONE',  ( -29.11475894678043730, -287.4258740215034322, -343.5937964168320491 ) ) ;
#35030=CARTESIAN_POINT ( 'NONE',  ( -11.89098930267787146, -290.6277527739537732, -200.8065911664070597 ) ) ;
#35031=CARTESIAN_POINT ( 'NONE',  ( 32.69712346968345429, -289.0485376442100005, -292.4779092497420265 ) ) ;
#35032=CARTESIAN_POINT ( 'NONE',  ( 10.59707575819634329, -289.1948066931273615, -210.1954327657594490 ) ) ;
#35033=CARTESIAN_POINT ( 'NONE',  ( -110.6895420685528819, -292.7540674466096675, -254.6449255276718588 ) ) ;
#35034=CARTESIAN_POINT ( 'NONE',  ( -105.5850139170171929, -288.9663577048036132, -238.7272238775061055 ) ) ;
#35035=CARTESIAN_POINT ( 'NONE',  ( -110.7372182995887897, -292.7511992959705367, -254.8698763474712621 ) ) ;
#35036=CARTESIAN_POINT ( 'NONE',  ( -70.09839522211105134, -286.5509159312609313, -204.8459266482407202 ) ) ;
#35037=CARTESIAN_POINT ( 'NONE',  ( -22.57938188942921087, -294.2407228061202886, -196.6052906834899829 ) ) ;
#35040=CARTESIAN_POINT ( 'NONE',  ( 22.31491323200852506, -276.9039361497368077, -224.3021467622433249 ) ) ;
#35041=CARTESIAN_POINT ( 'NONE',  ( -102.1415986314595443, -282.0475739677020783, -308.1231862601117655 ) ) ;
#35042=CARTESIAN_POINT ( 'NONE',  ( -112.4404954440458226, -295.9538031667455016, -254.0415229095897587 ) ) ;
#35043=CARTESIAN_POINT ( 'NONE',  ( 23.12142240598065968, -273.2041087588997357, -227.6521132108448171 ) ) ;
#35044=CARTESIAN_POINT ( 'NONE',  ( -103.4231509686823927, -277.0904095311445872, -235.9772063905259358 ) ) ;
#35045=CARTESIAN_POINT ( 'NONE',  ( -29.96513750278331401, -275.3526743908157641, -197.3356646905856167 ) ) ;
#35046=CARTESIAN_POINT ( 'NONE',  ( -66.26817020021830729, -296.8637195194720562, -338.0267240711888803 ) ) ;
#35048=CARTESIAN_POINT ( 'NONE',  ( -96.23637586860564852, -297.9622066296504954, -226.9346773168308857 ) ) ;
#35049=CARTESIAN_POINT ( 'NONE',  ( -15.85773043032068941, -284.3486647624100669, -198.0791666224836547 ) ) ;
#35050=CARTESIAN_POINT ( 'NONE',  ( -81.06930966476510037, -273.2729221968295406, -211.8434672281357223 ) ) ;
#35051=CARTESIAN_POINT ( 'NONE',  ( 27.13775883476131767, -286.9992249885727347, -228.2731224035461821 ) ) ;
#35052=CARTESIAN_POINT ( 'NONE',  ( -54.50103321318048444, -288.9333890928223809, -345.4578141987332174 ) ) ;
#35053=CARTESIAN_POINT ( 'NONE',  ( -94.32091129092921733, -297.8512790533748102, -319.6741618999815273 ) ) ;
#35054=CARTESIAN_POINT ( 'NONE',  ( -6.020196105746181026, -292.6393662886162019, -338.3242831247117692 ) ) ;
#35055=CARTESIAN_POINT ( 'NONE',  ( -39.57230616453448846, -279.2220148780185696, -193.5419540422863065 ) ) ;
#35056=CARTESIAN_POINT ( 'NONE',  ( -106.6662871844225293, -293.6237833571632336, -303.7098442033569654 ) ) ;
#35058=CARTESIAN_POINT ( 'NONE',  ( -45.42131696010972064, -287.9517222505797918, -343.3121309732811142 ) ) ;
#35060=CARTESIAN_POINT ( 'NONE',  ( -26.20232545359602128, -286.9103189074242550, -344.5817177250585246 ) ) ;
#35061=CARTESIAN_POINT ( 'NONE',  ( -102.6538186299615063, -274.5337074681983722, -236.1179301645551618 ) ) ;
#35062=CARTESIAN_POINT ( 'NONE',  ( -61.87575396307633468, -281.1647866547999683, -197.9403574164294639 ) ) ;
#35063=CARTESIAN_POINT ( 'NONE',  ( -105.6854468564162772, -294.1571668150403411, -302.1028741232273660 ) ) ;
#35064=CARTESIAN_POINT ( 'NONE',  ( 26.85504930592198747, -282.0263341306159077, -305.1142093861718081 ) ) ;
#35065=CARTESIAN_POINT ( 'NONE',  ( -98.27315770537690298, -296.0904225430992938, -317.4393240023110820 ) ) ;
#35066=CARTESIAN_POINT ( 'NONE',  ( -104.9280105224108723, -274.3670090560657968, -241.1206460327117327 ) ) ;
#35067=CARTESIAN_POINT ( 'NONE',  ( 9.552133459559023265, -282.6968129675674390, -211.7627926796758402 ) ) ;
#35068=CARTESIAN_POINT ( 'NONE',  ( -97.38312987122002085, -295.0280845433547370, -312.2948175903156880 ) ) ;
#35073=CARTESIAN_POINT ( 'NONE',  ( -72.15412193862135837, -285.4949136495443440, -336.3909755689485905 ) ) ;
#35075=CARTESIAN_POINT ( 'NONE',  ( 21.27581636871891391, -291.6952119285919025, -317.1477375740089997 ) ) ;
#35076=CARTESIAN_POINT ( 'NONE',  ( 25.92809382574244381, -275.3272183865963711, -314.0547070106519527 ) ) ;
#35077=CARTESIAN_POINT ( 'NONE',  ( 26.23559892921718273, -292.8931972852217882, -234.3841342450033665 ) ) ;
#35079=CARTESIAN_POINT ( 'NONE',  ( 29.95544662441509942, -283.4743252330021619, -300.5165012843273189 ) ) ;
#35080=CARTESIAN_POINT ( 'NONE',  ( -3.482472231383599404, -278.1974927048348150, -335.9354506382227328 ) ) ;
#35081=CARTESIAN_POINT ( 'NONE',  ( -41.51863522020822472, -284.5289162565445622, -346.7095682255419433 ) ) ;
#35082=CARTESIAN_POINT ( 'NONE',  ( 1.297366187555715200, -281.3188258148346108, -332.8236077957297994 ) ) ;
#35083=CARTESIAN_POINT ( 'NONE',  ( -82.51219249051763427, -281.4358380443744068, -210.4241328578222578 ) ) ;
#35084=CARTESIAN_POINT ( 'NONE',  ( -33.33448420970651682, -298.1010253735603328, -193.3611178742239929 ) ) ;
#35085=CARTESIAN_POINT ( 'NONE',  ( -3.996769887463077708, -276.4578096550213786, -339.7810603579957274 ) ) ;
#35086=CARTESIAN_POINT ( 'NONE',  ( 35.62320029464395787, -295.2815483374096175, -255.6153556392803523 ) ) ;
#35089=CARTESIAN_POINT ( 'NONE',  ( -65.17218556482481517, -293.5515436169272903, -340.8433304976075533 ) ) ;
#35090=CARTESIAN_POINT ( 'NONE',  ( 13.76990258603644435, -275.8198561066093362, -322.6387783478787128 ) ) ;
#35091=CARTESIAN_POINT ( 'NONE',  ( 17.08075998302576082, -295.8138976143769128, -323.9237076688007733 ) ) ;
#35092=CARTESIAN_POINT ( 'NONE',  ( 10.95989748297938249, -295.6061837355654234, -329.8850521119557584 ) ) ;
#35094=CARTESIAN_POINT ( 'NONE',  ( 29.88565193514773100, -289.9866415613514619, -303.2322536174998504 ) ) ;
#35095=CARTESIAN_POINT ( 'NONE',  ( -59.76808878727397456, -275.3431944365568711, -341.7549938832565886 ) ) ;
#35096=CARTESIAN_POINT ( 'NONE',  ( -57.52671180489815583, -281.7097081190568133, -198.7100223950835414 ) ) ;
#35097=CARTESIAN_POINT ( 'NONE',  ( -66.64201862571009372, -293.5188337672774423, -338.7921455630880700 ) ) ;
#35098=CARTESIAN_POINT ( 'NONE',  ( 26.79292985761020418, -282.8746400808794306, -229.9260790366863603 ) ) ;
#35099=CARTESIAN_POINT ( 'NONE',  ( -22.38338496074521444, -285.1683966839905793, -198.5422064699684199 ) ) ;
#35100=CARTESIAN_POINT ( 'NONE',  ( -81.88695342447972791, -220.3879184236133995, -351.6809530069663765 ) ) ;
#35102=CARTESIAN_POINT ( 'NONE',  ( -110.0150175914611879, -284.3193273053618100, -262.7436277951209718 ) ) ;
#35104=CARTESIAN_POINT ( 'NONE',  ( 24.86464926190132729, -283.2291745764003963, -315.2372064562601395 ) ) ;
#35105=CARTESIAN_POINT ( 'NONE',  ( -78.29714740122767580, -284.3090852276297937, -205.6258103314299603 ) ) ;
#35106=CARTESIAN_POINT ( 'NONE',  ( -73.66491904115208911, -280.5233534871238135, -202.7189689908636296 ) ) ;
#35107=CARTESIAN_POINT ( 'NONE',  ( -59.44551037914906289, -278.8534163515661817, -343.3962418862936374 ) ) ;
#35108=CARTESIAN_POINT ( 'NONE',  ( -92.05005921254146983, -298.4090924074129703, -314.0302885647153062 ) ) ;
#35109=CARTESIAN_POINT ( 'NONE',  ( -77.03173369861616493, -209.0939622114285896, -357.2395138152388654 ) ) ;
#35110=CARTESIAN_POINT ( 'NONE',  ( 1.543904745177172577, -276.5734098270466461, -206.4241321320548934 ) ) ;
#35111=CARTESIAN_POINT ( 'NONE',  ( -78.32199257516948876, -208.3160289898351039, -357.0357957823813990 ) ) ;
#35112=CARTESIAN_POINT ( 'NONE',  ( -92.49551339617238455, -277.2776776924193882, -220.0629700480870383 ) ) ;
#35113=CARTESIAN_POINT ( 'NONE',  ( -64.05385495817891695, -293.4687306080232361, -199.1689434712971547 ) ) ;
#35114=CARTESIAN_POINT ( 'NONE',  ( 16.22819808353040472, -293.6146896561054405, -320.1020334733168511 ) ) ;
#35115=CARTESIAN_POINT ( 'NONE',  ( -70.61813494197815544, -288.9868327067813425, -339.7456567375499503 ) ) ;
#35117=CARTESIAN_POINT ( 'NONE',  ( -44.75665195231122340, -293.7188518064703544, -346.4642630769265566 ) ) ;
#35118=CARTESIAN_POINT ( 'NONE',  ( -10.43956925982369022, -284.8089592220474628, -201.6254240591889868 ) ) ;
#35119=CARTESIAN_POINT ( 'NONE',  ( -34.83897387912438859, -293.9443433434321946, -196.1681139736239743 ) ) ;
#35120=CARTESIAN_POINT ( 'NONE',  ( -32.09388494005224146, -284.2997450642483841, -343.6666697104413402 ) ) ;
#35122=CARTESIAN_POINT ( 'NONE',  ( -40.63436127924891395, -292.9529698175599606, -193.6539177215897212 ) ) ;
#35123=CARTESIAN_POINT ( 'NONE',  ( -2.393716854173553177, -283.0688945432116839, -334.5363652291671315 ) ) ;
#35124=CARTESIAN_POINT ( 'NONE',  ( 25.38066613028506779, -292.9318826505336801, -314.3602872926184659 ) ) ;
#35125=CARTESIAN_POINT ( 'NONE',  ( 34.92410261474422839, -288.6871812556929626, -296.6275207227560031 ) ) ;
#35126=CARTESIAN_POINT ( 'NONE',  ( -46.01260315750639762, -289.6515226236320473, -346.8625005907836112 ) ) ;
#35127=CARTESIAN_POINT ( 'NONE',  ( 27.65717319731061252, -287.2660356853135113, -237.0209720823233113 ) ) ;
#35130=CARTESIAN_POINT ( 'NONE',  ( -112.8911560229499713, -298.4934431435319766, -263.9981615028202100 ) ) ;
#35131=CARTESIAN_POINT ( 'NONE',  ( -46.05696478967565355, -296.6286373044244442, -194.3522866930171062 ) ) ;
#35132=CARTESIAN_POINT ( 'NONE',  ( -93.79504581237952721, -276.9514881447387324, -317.0329754559917319 ) ) ;
#35133=CARTESIAN_POINT ( 'NONE',  ( -34.09950839995164529, -273.5995606539274263, -193.4909996258856495 ) ) ;
#35134=CARTESIAN_POINT ( 'NONE',  ( -31.56715743719263401, -293.4579460093494276, -343.8784509056085312 ) ) ;
#35135=CARTESIAN_POINT ( 'NONE',  ( 34.48726678029306925, -277.0799869147350023, -252.5124897734706906 ) ) ;
#35136=CARTESIAN_POINT ( 'NONE',  ( -44.64710468268618371, -296.1984390029592760, -196.6581185529536810 ) ) ;
#35137=CARTESIAN_POINT ( 'NONE',  ( -36.97825240356964827, -296.2525467787077105, -343.7697843894578682 ) ) ;
#35138=CARTESIAN_POINT ( 'NONE',  ( -9.099141060038419937, -295.7536331495725790, -338.0252367568480167 ) ) ;
#35140=CARTESIAN_POINT ( 'NONE',  ( -100.9491180487112985, -297.5936488349601063, -312.4152583790274207 ) ) ;
#35142=CARTESIAN_POINT ( 'NONE',  ( -111.4021019463929321, -294.3836093643077447, -283.5043596144729463 ) ) ;
#35143=CARTESIAN_POINT ( 'NONE',  ( 19.28711480348925278, -299.3951234332541844, -193.4569588003669480 ) ) ;
#35144=CARTESIAN_POINT ( 'NONE',  ( -85.08096386428900360, -288.3006753530420951, -326.4314056935131134 ) ) ;
#35145=CARTESIAN_POINT ( 'NONE',  ( -99.51505065204536038, -275.1208352737113501, -228.3223241137231128 ) ) ;
#35146=CARTESIAN_POINT ( 'NONE',  ( -90.12520477952683962, -273.8225208782365598, -214.3113218752585567 ) ) ;
#35148=CARTESIAN_POINT ( 'NONE',  ( -110.0717798650315871, -296.9785320766644645, -263.3018313253784299 ) ) ;
#35150=CARTESIAN_POINT ( 'NONE',  ( -12.08491086282274374, -282.3589573431759163, -199.3098510257975136 ) ) ;
#35151=CARTESIAN_POINT ( 'NONE',  ( 37.93730943332821681, -280.4097316369652049, -284.0855016050799122 ) ) ;
#35153=CARTESIAN_POINT ( 'NONE',  ( -86.04422592025551353, -283.0557899326468601, -329.8705858656843475 ) ) ;
#35154=CARTESIAN_POINT ( 'NONE',  ( 20.73780776296399253, -275.5829070763356867, -320.7802861776054328 ) ) ;
#35155=CARTESIAN_POINT ( 'NONE',  ( 5.748816988850379950, -279.0254450419402019, -207.5148949581167130 ) ) ;
#35156=CARTESIAN_POINT ( 'NONE',  ( -56.07453365475736717, -277.8114028518803025, -197.5124507396807303 ) ) ;
#35157=CARTESIAN_POINT ( 'NONE',  ( -32.63536286361777883, -272.6873203851653216, -196.9099087985494805 ) ) ;
#35158=CARTESIAN_POINT ( 'NONE',  ( -28.04941198657036239, -276.1701406127610881, -195.8876971949641472 ) ) ;
#35160=CARTESIAN_POINT ( 'NONE',  ( -102.9632401559879327, -295.2983825482343718, -231.9457594866861143 ) ) ;
#35161=CARTESIAN_POINT ( 'NONE',  ( -36.37361661899084453, -290.0843460592308247, -194.9993779147926318 ) ) ;
#35162=CARTESIAN_POINT ( 'NONE',  ( -50.56635501534110233, -291.8877222276124144, -194.5052777122625685 ) ) ;
#35163=CARTESIAN_POINT ( 'NONE',  ( 11.53235252346953921, -278.3760872149321699, -327.4693958504727789 ) ) ;
#35164=CARTESIAN_POINT ( 'NONE',  ( -18.75191855850065537, -272.2912262481341372, -197.6476279402562568 ) ) ;
#35166=CARTESIAN_POINT ( 'NONE',  ( -63.39217505487197712, -285.3091256307062622, -341.2884537110950305 ) ) ;
#35168=CARTESIAN_POINT ( 'NONE',  ( -41.47493295815851155, -283.9999627594650633, -195.4624494402378616 ) ) ;
#35170=CARTESIAN_POINT ( 'NONE',  ( -4.170862989313587121, -293.3996702235468206, -335.8490490180525399 ) ) ;
#35171=CARTESIAN_POINT ( 'NONE',  ( -1.570734421161609218, -284.6708018781619671, -205.2549634704404014 ) ) ;
#35173=CARTESIAN_POINT ( 'NONE',  ( -59.00974585222409274, -293.3323655896919036, -342.1629037603699430 ) ) ;
#35174=CARTESIAN_POINT ( 'NONE',  ( -112.4579771270189639, -282.8589345309415535, -284.0774599851088169 ) ) ;
#35175=CARTESIAN_POINT ( 'NONE',  ( -19.35913294916303684, -281.8873589836982774, -198.7326508194230712 ) ) ;
#35176=CARTESIAN_POINT ( 'NONE',  ( -54.88863481883083040, -287.0364732816289006, -195.7949473659950002 ) ) ;
#35177=CARTESIAN_POINT ( 'NONE',  ( 20.81974377915599206, -280.4592680848270447, -319.2612249246336091 ) ) ;
#35178=CARTESIAN_POINT ( 'NONE',  ( 33.71031196159538013, -287.3304598633699811, -253.5556297796739500 ) ) ;
#35179=CARTESIAN_POINT ( 'NONE',  ( -89.49067187255319311, -279.2296081869910154, -322.3551283074796743 ) ) ;
#35180=CARTESIAN_POINT ( 'NONE',  ( -107.7765413463411193, -279.6165134930624845, -250.5274217184221186 ) ) ;
#35181=CARTESIAN_POINT ( 'NONE',  ( -98.03480622130315680, -287.1393108790977067, -225.6125606721149666 ) ) ;
#35183=CARTESIAN_POINT ( 'NONE',  ( -103.8487329771342900, -296.8915871200160836, -231.4512189537137772 ) ) ;
#35184=CARTESIAN_POINT ( 'NONE',  ( 37.27532521466388715, -289.5765603476536398, -273.8112632980647163 ) ) ;
#35186=CARTESIAN_POINT ( 'NONE',  ( -72.08107566293803359, -276.1233781216987495, -198.2974183793908196 ) ) ;
#35188=CARTESIAN_POINT ( 'NONE',  ( 8.414981144280172742, -272.6768079114083321, -210.7259392502402022 ) ) ;
#35189=CARTESIAN_POINT ( 'NONE',  ( 38.43919010718616391, -292.0590079796406826, -278.8264501444517123 ) ) ;
#35190=CARTESIAN_POINT ( 'NONE',  ( -90.08595122003215749, -296.7894884770489057, -219.7315038131477820 ) ) ;
#35191=CARTESIAN_POINT ( 'NONE',  ( 34.38066818839624261, -288.8503355149758249, -253.3770917654753418 ) ) ;
#35192=CARTESIAN_POINT ( 'NONE',  ( 17.80305468640262845, -282.6156393282927866, -220.9948336274530902 ) ) ;
#35193=CARTESIAN_POINT ( 'NONE',  ( -70.36783672594074801, -290.9041416471278012, -339.2803579258600735 ) ) ;
#35194=CARTESIAN_POINT ( 'NONE',  ( -111.7789606448097146, -291.6441437160613077, -288.0917515122961845 ) ) ;
#35195=CARTESIAN_POINT ( 'NONE',  ( -107.0640408638667509, -286.1908228931040981, -298.1392233310317010 ) ) ;
#35196=CARTESIAN_POINT ( 'NONE',  ( -113.0652416208005633, -278.5433079883870278, -284.3958294107782194 ) ) ;
#35198=CARTESIAN_POINT ( 'NONE',  ( -0.1892511644907210466, -292.6418881540054144, -336.1712218482339267 ) ) ;
#35199=CARTESIAN_POINT ( 'NONE',  ( 38.42518934517773488, -281.5580400392859133, -284.1594466030773560 ) ) ;
#35200=CARTESIAN_POINT ( 'NONE',  ( -51.82526126042856163, -275.7254368878644755, -197.4998507447658653 ) ) ;
#35202=CARTESIAN_POINT ( 'NONE',  ( -6.998514795304313196, -282.9805209788415823, -207.2794874003663779 ) ) ;
#35203=CARTESIAN_POINT ( 'NONE',  ( -4.453982600200022013, -274.8646064966455924, -338.8763144015833859 ) ) ;
#35205=AXIS2_PLACEMENT_3D ( 'NONE', #60773, #15825, #80669 ) ;
#35206=CARTESIAN_POINT ( 'NONE',  ( 26.90618844118116826, -281.5340661876780928, -305.1490074827225385 ) ) ;
#35208=CARTESIAN_POINT ( 'NONE',  ( -88.93330921929572241, -278.9633320578240614, -326.9854465793111444 ) ) ;
#35209=CARTESIAN_POINT ( 'NONE',  ( -91.49718789812359887, -274.5757289615240211, -220.6592207342119423 ) ) ;
#35210=CARTESIAN_POINT ( 'NONE',  ( -52.11622030124287619, -284.9263514514747158, -194.9773944654879756 ) ) ;
#35211=CARTESIAN_POINT ( 'NONE',  ( -94.87807847671112427, -291.6627561658496575, -316.9179561813990631 ) ) ;
#35212=CARTESIAN_POINT ( 'NONE',  ( -110.2774149309257723, -274.4342014711707520, -248.1165464941674088 ) ) ;
#35214=CARTESIAN_POINT ( 'NONE',  ( -15.93152513608725052, -275.6384655142044835, -196.8561362936036687 ) ) ;
#35216=CARTESIAN_POINT ( 'NONE',  ( -100.2612980934016917, -298.0042605506891960, -310.9671402915281533 ) ) ;
#35217=CARTESIAN_POINT ( 'NONE',  ( -107.9109168409701596, -282.2269498383935797, -295.4156600920512119 ) ) ;
#35219=CARTESIAN_POINT ( 'NONE',  ( -113.7930766539588348, -290.1008250370772430, -279.7974675758250100 ) ) ;
#35220=CARTESIAN_POINT ( 'NONE',  ( 35.73669741397215205, -273.3752093012220712, -255.0869582807416407 ) ) ;
#35221=CARTESIAN_POINT ( 'NONE',  ( -2.605959168264249559, -288.1038210257819401, -202.5241882912712867 ) ) ;
#35222=CARTESIAN_POINT ( 'NONE',  ( -105.4051403116671679, -289.1079206582259644, -297.7296520166478331 ) ) ;
#35224=CARTESIAN_POINT ( 'NONE',  ( -94.26017601693298786, -289.8237752516374144, -219.3817751469406971 ) ) ;
#35225=CARTESIAN_POINT ( 'NONE',  ( -99.72747028583918905, -290.7413698035805965, -232.4124267198380949 ) ) ;
#35227=CARTESIAN_POINT ( 'NONE',  ( 39.33071437110933033, -288.6106856601679169, -268.6778581246182398 ) ) ;
#35228=CARTESIAN_POINT ( 'NONE',  ( -87.10684196784009714, -278.1020191509133497, -323.7981664075922481 ) ) ;
#35230=CARTESIAN_POINT ( 'NONE',  ( 15.25665350483664540, -293.2502009538767425, -326.1724582659211364 ) ) ;
#35231=CARTESIAN_POINT ( 'NONE',  ( -24.54236882900957539, -283.5444587441600675, -346.2405541171568188 ) ) ;
#35232=CARTESIAN_POINT ( 'NONE',  ( -60.50760296608934397, -286.0931184365711033, -196.8951669331631251 ) ) ;
#35233=CARTESIAN_POINT ( 'NONE',  ( -29.43814751788083584, -283.2827070557685261, -343.0037939215443998 ) ) ;
#35234=CARTESIAN_POINT ( 'NONE',  ( -78.06300626195221071, -208.5067154030725476, -357.1885865629087107 ) ) ;
#35235=CARTESIAN_POINT ( 'NONE',  ( -40.80092957519016039, -139.0259249319638002, -363.6696181199743023 ) ) ;
#35236=CARTESIAN_POINT ( 'NONE',  ( 159.7936134115024345, 218.3991897550104966, -202.4342046892747078 ) ) ;
#35237=CARTESIAN_POINT ( 'NONE',  ( -110.5031764828875396, -271.7494487804054302, -270.3509199023655469 ) ) ;
#35238=CARTESIAN_POINT ( 'NONE',  ( -35.36828291736804175, -272.9977917035798782, -197.0660128374298665 ) ) ;
#35239=CARTESIAN_POINT ( 'NONE',  ( -34.86291060757183402, -294.5294485291665296, -347.2596388131365757 ) ) ;
#35240=CARTESIAN_POINT ( 'NONE',  ( 161.7159580759288815, 217.5486918941278418, -202.6611147385943354 ) ) ;
#35241=CARTESIAN_POINT ( 'NONE',  ( -27.04619406426520811, -272.8651210279446104, -194.4970748072591107 ) ) ;
#35242=CARTESIAN_POINT ( 'NONE',  ( -110.0905285846461226, -298.2200096415716644, -285.2051726285597510 ) ) ;
#35243=CARTESIAN_POINT ( 'NONE',  ( -37.56463551181180094, -293.1290060949550025, -197.0398476178612555 ) ) ;
#35246=CARTESIAN_POINT ( 'NONE',  ( -100.5637074175163832, -298.0702343856254402, -226.7972501618737624 ) ) ;
#35247=CARTESIAN_POINT ( 'NONE',  ( 22.01534606782081127, -288.6395021693905392, -312.9607601015925979 ) ) ;
#35249=CARTESIAN_POINT ( 'NONE',  ( 39.44588811497572323, -294.3900413975638912, -273.1584581180337068 ) ) ;
#35250=CARTESIAN_POINT ( 'NONE',  ( -39.10014349113041732, -295.5660103188100720, -347.2794823723841660 ) ) ;
#35251=CARTESIAN_POINT ( 'NONE',  ( 34.90743487784244792, -293.5810685688406352, -259.9178189155641121 ) ) ;
#35253=CARTESIAN_POINT ( 'NONE',  ( 35.88356750541262841, -277.2346337947118968, -251.7231357639323903 ) ) ;
#35255=CARTESIAN_POINT ( 'NONE',  ( -113.7059633698434880, -277.9370919454821660, -280.1654332635939113 ) ) ;
#35256=CARTESIAN_POINT ( 'NONE',  ( 35.87790370661325312, -276.4734764132098235, -268.8451820742031941 ) ) ;
#35257=CARTESIAN_POINT ( 'NONE',  ( -36.96753129560219975, -275.8169428051940599, -194.3624893066706534 ) ) ;
#35258=CARTESIAN_POINT ( 'NONE',  ( 36.56417227919467194, -273.7602237509616430, -285.0692391952514413 ) ) ;
#35259=CARTESIAN_POINT ( 'NONE',  ( -110.3145313817427109, -297.2607761888939990, -266.0184728521508646 ) ) ;
#35260=CARTESIAN_POINT ( 'NONE',  ( -109.0471243335262415, -295.3433759139555832, -253.8170236080210032 ) ) ;
#35262=CARTESIAN_POINT ( 'NONE',  ( -93.03354370565018883, -279.7715123087858160, -217.2006664199690249 ) ) ;
#35263=CARTESIAN_POINT ( 'NONE',  ( -16.37883840391437573, -276.9403619103208598, -340.3395050251974112 ) ) ;
#35264=CARTESIAN_POINT ( 'NONE',  ( 39.14738155672085185, -286.2162256951568793, -268.7122837099698813 ) ) ;
#35265=CARTESIAN_POINT ( 'NONE',  ( -111.8779441903994751, -274.6592404277505466, -262.0335151623966681 ) ) ;
#35268=CARTESIAN_POINT ( 'NONE',  ( 34.15598294770959598, -286.5451143551745190, -254.8471551645389752 ) ) ;
#35269=CARTESIAN_POINT ( 'NONE',  ( -65.17671216468951911, -277.9231930766616756, -201.7813387523666790 ) ) ;
#35270=CARTESIAN_POINT ( 'NONE',  ( -101.3151644604992896, -277.6210199222451251, -233.9912021565911289 ) ) ;
#35271=CARTESIAN_POINT ( 'NONE',  ( -98.74513084906185156, -287.1372543737727483, -227.2736937462622393 ) ) ;
#35272=CARTESIAN_POINT ( 'NONE',  ( -51.34167688163601895, -278.4402474850571139, -342.4106228704139312 ) ) ;
#35275=CARTESIAN_POINT ( 'NONE',  ( -62.09732662507806822, -275.6094125554237735, -342.2577171105186267 ) ) ;
#35277=CARTESIAN_POINT ( 'NONE',  ( -2.872912963869989955, -275.1719479777118522, -205.8956591705210144 ) ) ;
#35278=CARTESIAN_POINT ( 'NONE',  ( 16.53053704046080696, -284.2891632778894859, -322.8550797438385302 ) ) ;
#35280=CARTESIAN_POINT ( 'NONE',  ( 17.61458404037442804, -290.1939152879416497, -322.2178535949965976 ) ) ;
#35282=CARTESIAN_POINT ( 'NONE',  ( -45.46885936090239966, -289.9491379481171407, -195.7516741655833812 ) ) ;
#35284=CARTESIAN_POINT ( 'NONE',  ( -1.467369808913267848, -273.2232015027394141, -206.2040847470133542 ) ) ;
#35285=CARTESIAN_POINT ( 'NONE',  ( 13.77048810584812877, -290.9175361705032969, -216.5242375703555240 ) ) ;
#35286=CARTESIAN_POINT ( 'NONE',  ( 198.7213489544213303, 274.9184959104715631, -125.0903475807052416 ) ) ;
#35288=CARTESIAN_POINT ( 'NONE',  ( -31.89576399111479432, -287.4646290104125796, -346.5252862749107976 ) ) ;
#35289=CARTESIAN_POINT ( 'NONE',  ( -78.80950385535176395, -285.2215242630711032, -331.4091455325706193 ) ) ;
#35290=CARTESIAN_POINT ( 'NONE',  ( 2.232645568271720560, -284.8144243973138714, -205.4932123914291537 ) ) ;
#35292=CARTESIAN_POINT ( 'NONE',  ( -85.23159774975364655, -285.1543755263406865, -326.2353752154668882 ) ) ;
#35293=CARTESIAN_POINT ( 'NONE',  ( -40.23052178807429158, -283.8922255226194693, -343.4655394408608231 ) ) ;
#35294=CARTESIAN_POINT ( 'NONE',  ( -111.7322060136481667, -292.3784462725532194, -282.3802459801327700 ) ) ;
#35295=CARTESIAN_POINT ( 'NONE',  ( 7.368925629068237448, -274.5281663898666125, -331.3379027065130913 ) ) ;
#35296=CARTESIAN_POINT ( 'NONE',  ( 25.30722190772271318, -275.2924921395457432, -225.6076313383064189 ) ) ;
#35298=CARTESIAN_POINT ( 'NONE',  ( -101.0995803351279676, -288.0892729156792029, -311.0067632723485644 ) ) ;
#35299=CARTESIAN_POINT ( 'NONE',  ( -25.76996866147937126, -276.9086265280614043, -346.4866395299678743 ) ) ;
#35300=CARTESIAN_POINT ( 'NONE',  ( -23.18267267301051149, -296.8502258103880536, -343.7035100873140436 ) ) ;
#35303=CARTESIAN_POINT ( 'NONE',  ( -91.11362499387101366, -282.5214086041353880, -320.4592574139649059 ) ) ;
#35304=CARTESIAN_POINT ( 'NONE',  ( -28.43652130149055779, -278.1648302356249474, -195.8394381513753046 ) ) ;
#35306=CARTESIAN_POINT ( 'NONE',  ( -103.6176530311758768, -271.5289067674997909, -232.4370613619283006 ) ) ;
#35307=CARTESIAN_POINT ( 'NONE',  ( -106.3631949085399526, -277.5790271343043969, -294.5963379074660224 ) ) ;
#35308=CARTESIAN_POINT ( 'NONE',  ( 16.68044971575040947, -295.7858743692547705, -320.4841174841319003 ) ) ;
#35310=CARTESIAN_POINT ( 'NONE',  ( 17.01377030590352746, -279.7248184309614771, -216.1851107612656335 ) ) ;
#35311=CARTESIAN_POINT ( 'NONE',  ( 31.76606354608881588, -294.8166633918522734, -294.7519593685512973 ) ) ;
#35312=CARTESIAN_POINT ( 'NONE',  ( -95.19752181008296077, -297.1866683211546274, -320.4211037123490655 ) ) ;
#35313=CARTESIAN_POINT ( 'NONE',  ( -57.90274796562979276, -297.6123617108498252, -200.3165370621973977 ) ) ;
#35314=CARTESIAN_POINT ( 'NONE',  ( -51.09386068274324799, -291.2279474034933742, -344.1426212696375728 ) ) ;
#35315=CARTESIAN_POINT ( 'NONE',  ( -26.62320554959377006, -286.3514578286117853, -194.0572822414794416 ) ) ;
#35316=CARTESIAN_POINT ( 'NONE',  ( -41.10728688480014625, -272.1449585913027249, -194.6385265679608949 ) ) ;
#35317=CARTESIAN_POINT ( 'NONE',  ( 38.02394462383258400, -287.1873193955063925, -254.5169133978125160 ) ) ;
#35318=CARTESIAN_POINT ( 'NONE',  ( -37.02612016570056142, -282.0360135039760507, -195.7169807954790883 ) ) ;
#35320=CARTESIAN_POINT ( 'NONE',  ( -95.13537540735848097, -284.2428779053269636, -225.3596569305279615 ) ) ;
#35321=CARTESIAN_POINT ( 'NONE',  ( -56.79729785548920518, -287.3027138213166154, -342.8473892216402987 ) ) ;
#35322=CARTESIAN_POINT ( 'NONE',  ( 61.48257290429442889, 47.14312216093964025, -312.8229988924202871 ) ) ;
#35323=CARTESIAN_POINT ( 'NONE',  ( -27.82233136360427750, -285.6839534929694082, -197.9223848359166027 ) ) ;
#35324=CARTESIAN_POINT ( 'NONE',  ( 30.87355905880138707, -282.9485999712395596, -305.5676319588594083 ) ) ;
#35325=CARTESIAN_POINT ( 'NONE',  ( -111.3184403234689483, -289.3532816506603353, -290.8614136740770277 ) ) ;
#35326=CARTESIAN_POINT ( 'NONE',  ( -68.36566886428350642, -281.2515098213852980, -200.7483611714270637 ) ) ;
#35327=CARTESIAN_POINT ( 'NONE',  ( -99.04016210309333701, -280.4722264883238836, -225.0996595195135512 ) ) ;
#35328=CARTESIAN_POINT ( 'NONE',  ( 21.00862402647616989, -282.0016731778902113, -314.2479301254109032 ) ) ;
#35329=CARTESIAN_POINT ( 'NONE',  ( 30.89540736609959382, -277.1423916892329657, -239.1116677640277999 ) ) ;
#35330=CARTESIAN_POINT ( 'NONE',  ( 24.02897609703129689, -294.1717096876017763, -316.8653124135184953 ) ) ;
#35331=CARTESIAN_POINT ( 'NONE',  ( -7.585482484714454188, -286.6803959945262932, -338.8737553279843837 ) ) ;
#35332=CARTESIAN_POINT ( 'NONE',  ( 38.80816098110800283, -295.1872088678599653, -273.1250041152688368 ) ) ;
#35333=CARTESIAN_POINT ( 'NONE',  ( -107.9040592593216417, -295.2108041010885131, -290.2402414033725222 ) ) ;
#35335=CARTESIAN_POINT ( 'NONE',  ( 35.64736362416090287, -283.6623426501461722, -285.0510579369343986 ) ) ;
#35336=CARTESIAN_POINT ( 'NONE',  ( -109.0656378708356158, -296.4004569082486569, -256.5918340760067622 ) ) ;
#35338=CARTESIAN_POINT ( 'NONE',  ( 21.96145215872486389, -293.9761660017497888, -221.7336705896772457 ) ) ;
#35339=CARTESIAN_POINT ( 'NONE',  ( -26.71977809016659933, -283.5650285303413511, -342.7386086586990928 ) ) ;
#35342=CARTESIAN_POINT ( 'NONE',  ( -55.26701246912546139, -272.8857476170014138, -195.7186140738851918 ) ) ;
#35343=CARTESIAN_POINT ( 'NONE',  ( -93.51265647848390472, -290.4857252523443663, -322.9558131065182351 ) ) ;
#35344=CARTESIAN_POINT ( 'NONE',  ( -21.99963323167070328, -280.9971832273852215, -344.5563096135813339 ) ) ;
#35345=CARTESIAN_POINT ( 'NONE',  ( -114.2299764661069759, -290.8387301814705665, -274.0943810606559623 ) ) ;
#35346=CARTESIAN_POINT ( 'NONE',  ( 35.29499233449146089, -287.7867479008825171, -262.8779104595309946 ) ) ;
#35350=CARTESIAN_POINT ( 'NONE',  ( 138.5936043815089249, 178.2952344932181461, -238.2260155999035192 ) ) ;
#35351=CARTESIAN_POINT ( 'NONE',  ( -37.30987171927208834, -271.5523547857346784, -195.3611179825600175 ) ) ;
#35352=CARTESIAN_POINT ( 'NONE',  ( -85.58300483283683491, -278.5614089002287983, -215.3576794820942553 ) ) ;
#35353=ORIENTED_EDGE ( 'NONE', *, *, #82664, .F. ) ;
#35354=CARTESIAN_POINT ( 'NONE',  ( -62.40174770981307972, -278.6387869451376673, -201.4147233026683068 ) ) ;
#35355=CARTESIAN_POINT ( 'NONE',  ( 39.35907415515357854, -275.3006515257243336, -276.8983586705458038 ) ) ;
#35356=CARTESIAN_POINT ( 'NONE',  ( -109.1495399033135385, -270.4770199085714921, -295.6887214991818382 ) ) ;
#35357=CARTESIAN_POINT ( 'NONE',  ( -113.7956355219171343, -277.1115102838527378, -271.5807374497644560 ) ) ;
#35359=CARTESIAN_POINT ( 'NONE',  ( -62.10361138193461983, -281.3956773573856935, -340.8335602679312615 ) ) ;
#35360=CARTESIAN_POINT ( 'NONE',  ( -89.99355683654316351, -297.5433521758166080, -325.2218215773887664 ) ) ;
#35362=CARTESIAN_POINT ( 'NONE',  ( 32.81102065386793498, -294.3147946737682332, -290.8164930270691571 ) ) ;
#35364=CARTESIAN_POINT ( 'NONE',  ( -94.66510066510163313, -289.8828471751627944, -224.3490475274149674 ) ) ;
#35365=CARTESIAN_POINT ( 'NONE',  ( -13.10249022103224270, -275.0104237766035453, -197.3832207158263259 ) ) ;
#35366=CARTESIAN_POINT ( 'NONE',  ( -37.82464763943075070, -298.2126168200189227, -197.3627154915492383 ) ) ;
#35374=CARTESIAN_POINT ( 'NONE',  ( -68.66780278378681146, -280.7100926693755127, -204.0821517331897326 ) ) ;
#35375=CARTESIAN_POINT ( 'NONE',  ( -20.00943296855395204, -282.0319375529127797, -196.3235165764820920 ) ) ;
#35376=CARTESIAN_POINT ( 'NONE',  ( -110.3312503004726608, -283.5320716230345397, -276.3556165693473758 ) ) ;
#35377=CARTESIAN_POINT ( 'NONE',  ( 1.018271775213363650, -282.4299549386903436, -206.7455215406967852 ) ) ;
#35378=CARTESIAN_POINT ( 'NONE',  ( 18.82440290605323341, -274.7040443977327300, -318.0693628042634487 ) ) ;
#35381=CARTESIAN_POINT ( 'NONE',  ( -77.72132687017663955, -278.3821887997426074, -335.7960623972807639 ) ) ;
#35386=CARTESIAN_POINT ( 'NONE',  ( -70.98135671140305192, -285.4737339476653801, -337.7909356585846012 ) ) ;
#35387=CARTESIAN_POINT ( 'NONE',  ( 34.37680400917464141, -292.5590021248916059, -255.9022835984209792 ) ) ;
#35388=CARTESIAN_POINT ( 'NONE',  ( -34.67866899794705660, -288.3681006042632475, -347.2130603918622569 ) ) ;
#35389=CARTESIAN_POINT ( 'NONE',  ( -52.27174511611867302, -284.0982131031319682, -197.8692717680117710 ) ) ;
#35390=CARTESIAN_POINT ( 'NONE',  ( -104.0116636951921265, -283.5456209448807954, -239.0876811960825705 ) ) ;
#35391=CARTESIAN_POINT ( 'NONE',  ( -87.43143793499899630, -288.0018076344250062, -324.9191241967814676 ) ) ;
#35392=CARTESIAN_POINT ( 'NONE',  ( -10.81803359171806456, -283.9036357956117627, -338.8520147168692347 ) ) ;
#35393=CARTESIAN_POINT ( 'NONE',  ( -36.92459258890065144, -272.0572502219812350, -195.3495599354373837 ) ) ;
#35394=CARTESIAN_POINT ( 'NONE',  ( -107.4986434170018015, -282.5679858648593381, -300.2357864277485078 ) ) ;
#35395=CARTESIAN_POINT ( 'NONE',  ( -71.14909938523703659, -297.4985909073644166, -337.3093099517820974 ) ) ;
#35396=CARTESIAN_POINT ( 'NONE',  ( -49.03381529791319338, -283.9034929611922848, -196.0569101383812267 ) ) ;
#35397=CARTESIAN_POINT ( 'NONE',  ( -102.0592721434700252, -279.0279633579047527, -304.6400374502080126 ) ) ;
#35398=CARTESIAN_POINT ( 'NONE',  ( 25.91604973283455493, -290.0990160655243812, -311.0586840981738987 ) ) ;
#35401=CARTESIAN_POINT ( 'NONE',  ( 38.16873689043865880, -295.5071830387250316, -273.0975566514466664 ) ) ;
#35402=CARTESIAN_POINT ( 'NONE',  ( -109.0358133292690752, -276.2660599902676495, -292.5569101221272490 ) ) ;
#35403=CARTESIAN_POINT ( 'NONE',  ( -111.7681878592238292, -289.5091854243160014, -289.5150058189582296 ) ) ;
#35404=CARTESIAN_POINT ( 'NONE',  ( -85.01020390609726007, -294.1222714751994545, -326.7678634916808278 ) ) ;
#35405=CARTESIAN_POINT ( 'NONE',  ( -39.70039309408342376, -278.7067698291309057, -196.8932206199147572 ) ) ;
#35406=CARTESIAN_POINT ( 'NONE',  ( -81.91406062905878116, -271.5197303448059074, -210.6758288227294997 ) ) ;
#35407=CARTESIAN_POINT ( 'NONE',  ( -5.845371623542153117, -293.7903173055038337, -203.9452511240053525 ) ) ;
#35408=CARTESIAN_POINT ( 'NONE',  ( -69.85430415644619018, -279.9805209788416391, -337.9475929042657754 ) ) ;
#35409=CARTESIAN_POINT ( 'NONE',  ( -4.815798806994362025, -293.1114493030560766, -339.4027942529838811 ) ) ;
#35410=CARTESIAN_POINT ( 'NONE',  ( -73.92400415662122271, -291.1467725700177311, -334.4707355352870763 ) ) ;
#35411=CARTESIAN_POINT ( 'NONE',  ( 12.62915964942925484, -290.9776741098256139, -213.1170162376579640 ) ) ;
#35413=CARTESIAN_POINT ( 'NONE',  ( 10.51209116820994538, -289.8016599912456286, -326.3336933605255012 ) ) ;
#35415=CARTESIAN_POINT ( 'NONE',  ( -70.03544029195215614, -290.2970748734683184, -335.8251484747642053 ) ) ;
#35417=CARTESIAN_POINT ( 'NONE',  ( -101.9580256934992946, -291.2139989372096238, -311.6016137616600759 ) ) ;
#35418=CARTESIAN_POINT ( 'NONE',  ( 36.64467246944092693, -279.3895479394639665, -256.0634442057819342 ) ) ;
#35419=CARTESIAN_POINT ( 'NONE',  ( -65.32695985371928771, -291.6759040720776284, -202.9248685316386798 ) ) ;
#35421=CARTESIAN_POINT ( 'NONE',  ( -50.93962971697916231, -279.8829872176186200, -194.5713013124071438 ) ) ;
#35422=CARTESIAN_POINT ( 'NONE',  ( 21.59108881676021596, -281.8858973652204440, -319.8855632474826507 ) ) ;
#35423=CARTESIAN_POINT ( 'NONE',  ( -6.162439755335780589, -284.4616492636437215, -202.1351779158216004 ) ) ;
#35424=CARTESIAN_POINT ( 'NONE',  ( 12.73271565463508992, -280.4842665362771186, -325.1645700833301476 ) ) ;
#35425=CARTESIAN_POINT ( 'NONE',  ( -94.28103874402968643, -283.2289695988396261, -221.4681694013947890 ) ) ;
#35426=CARTESIAN_POINT ( 'NONE',  ( -17.15659691235342876, -278.7880140560332052, -196.7726042104499413 ) ) ;
#35427=AXIS2_PLACEMENT_3D ( 'NONE', #26544, #61600, #70585 ) ;
#35428=CARTESIAN_POINT ( 'NONE',  ( 32.43651670737484949, -286.0626436911474002, -238.4135341959922130 ) ) ;
#35429=CARTESIAN_POINT ( 'NONE',  ( 33.98891344527550018, -276.1402358258592926, -254.0402931635526897 ) ) ;
#35431=CARTESIAN_POINT ( 'NONE',  ( -38.93505923740826802, -293.6319629735266403, -196.5783176565981307 ) ) ;
#35432=CARTESIAN_POINT ( 'NONE',  ( 38.33806485315447077, -276.8445348388815432, -259.8169506347200013 ) ) ;
#35433=CARTESIAN_POINT ( 'NONE',  ( -106.2855763294272151, -277.8971079005302158, -294.5733663795613779 ) ) ;
#35434=CARTESIAN_POINT ( 'NONE',  ( -77.17108033825789448, -291.7008577034122254, -204.4010627264145228 ) ) ;
#35436=CARTESIAN_POINT ( 'NONE',  ( -5.527616766370074153, -278.5472189395063651, -201.8251544180090775 ) ) ;
#35438=CARTESIAN_POINT ( 'NONE',  ( -69.62122395575467237, -291.4722118480507334, -200.4394641163905249 ) ) ;
#35439=CARTESIAN_POINT ( 'NONE',  ( -107.2225524608957130, -289.9008563869512614, -248.4082829704373125 ) ) ;
#35440=CARTESIAN_POINT ( 'NONE',  ( -63.59070751608000904, -293.3941268107629980, -340.6177209436892781 ) ) ;
#35444=CARTESIAN_POINT ( 'NONE',  ( -66.58295218394705728, -291.1661396866224436, -203.4063749092488820 ) ) ;
#35446=CARTESIAN_POINT ( 'NONE',  ( 17.36665895637873192, -273.6952119285918457, -314.0302885647153062 ) ) ;
#35447=CARTESIAN_POINT ( 'NONE',  ( -111.7435737959687145, -295.3730917661030162, -289.3134617385844081 ) ) ;
#35448=CARTESIAN_POINT ( 'NONE',  ( -93.06082709831257205, -285.1469095971032743, -322.8081474383906198 ) ) ;
#35449=CARTESIAN_POINT ( 'NONE',  ( -38.62277864818258166, -285.8689994018389484, -197.3598779483117767 ) ) ;
#35450=CARTESIAN_POINT ( 'NONE',  ( 29.70892005420766679, -276.6624304283904507, -239.6612491835425374 ) ) ;
#35451=CARTESIAN_POINT ( 'NONE',  ( -37.01307056537550011, -293.0680948198364604, -345.0179024847935239 ) ) ;
#35452=CARTESIAN_POINT ( 'NONE',  ( -109.5760164090117570, -298.1024255590058942, -286.4911386907660358 ) ) ;
#35454=CARTESIAN_POINT ( 'NONE',  ( 7.812662599335469693, -275.2149017442992545, -328.2896233777790940 ) ) ;
#35457=CARTESIAN_POINT ( 'NONE',  ( -79.46894210689021065, -295.2712311838648702, -334.7896813277532146 ) ) ;
#35458=CARTESIAN_POINT ( 'NONE',  ( -15.40439500297898689, -290.6862747222315306, -341.5491525112072395 ) ) ;
#35460=CARTESIAN_POINT ( 'NONE',  ( 25.78825877897586594, -288.7099537500333213, -307.3190575948840433 ) ) ;
#35462=CARTESIAN_POINT ( 'NONE',  ( -6.314446994652713308, -279.5086174983890714, -200.1320052817969213 ) ) ;
#35463=CARTESIAN_POINT ( 'NONE',  ( -16.52648650585935641, -295.4415855182214727, -344.4435695842685163 ) ) ;
#35464=CARTESIAN_POINT ( 'NONE',  ( -71.37322890248786678, -287.6363422902873594, -338.0527757644180156 ) ) ;
#35465=CARTESIAN_POINT ( 'NONE',  ( -113.7543057210643695, -297.0020208053404644, -261.0413541453291373 ) ) ;
#35466=CARTESIAN_POINT ( 'NONE',  ( 31.81969329244595812, -293.5723878375407025, -246.7774943301253927 ) ) ;
#35470=CARTESIAN_POINT ( 'NONE',  ( 18.15398598407957564, -289.7939477327786904, -322.7341699796975263 ) ) ;
#35471=CARTESIAN_POINT ( 'NONE',  ( -119.3990491898856732, -294.0523547857346784, -270.3284710469131937 ) ) ;
#35473=CARTESIAN_POINT ( 'NONE',  ( -82.17269701044327235, -278.8067737953701908, -207.8831658327532068 ) ) ;
#35474=CARTESIAN_POINT ( 'NONE',  ( -18.24377381170336676, -284.8057763897393784, -342.7702001993695831 ) ) ;
#35475=CARTESIAN_POINT ( 'NONE',  ( -37.95933222389735562, -284.6192906643012179, -193.9528407740463933 ) ) ;
#35476=CARTESIAN_POINT ( 'NONE',  ( 36.38320225558939569, -285.7663519917486497, -280.7470542302582430 ) ) ;
#35477=CARTESIAN_POINT ( 'NONE',  ( 25.06318338630315878, -277.9900370645592602, -313.4163189315645468 ) ) ;
#35480=CARTESIAN_POINT ( 'NONE',  ( -110.3919325758372594, -278.5484989262219528, -270.6380536738776641 ) ) ;
#35481=CARTESIAN_POINT ( 'NONE',  ( -51.83947225011938542, -279.2104355055322458, -198.6594224968718834 ) ) ;
#35482=CARTESIAN_POINT ( 'NONE',  ( -3.973080912198417636, -275.5616219418762398, -201.2957622270114655 ) ) ;
#35483=CARTESIAN_POINT ( 'NONE',  ( -110.9514180564329990, -277.6143165612652410, -249.1569168530786271 ) ) ;
#35484=CARTESIAN_POINT ( 'NONE',  ( 200.9738417244596178, 294.2968953162039156, -68.37162730693829360 ) ) ;
#35485=CARTESIAN_POINT ( 'NONE',  ( -92.00993445479919330, -274.2358724459490986, -216.4704474699857712 ) ) ;
#35486=ADVANCED_FACE ( 'NONE', ( #91973, #33761 ), #49373, .T. ) ;
#35488=CARTESIAN_POINT ( 'NONE',  ( -9.396827642807163983, -299.8208190870045655, -193.9437202937408813 ) ) ;
#35489=CARTESIAN_POINT ( 'NONE',  ( -95.99890600148557951, -281.6948066931273615, -223.6242672951989618 ) ) ;
#35491=CARTESIAN_POINT ( 'NONE',  ( -49.48621853281270688, -286.9734890362925626, -198.0132261012766719 ) ) ;
#35492=CARTESIAN_POINT ( 'NONE',  ( -46.40713285024969537, -287.6987542755727532, -194.9171524050337041 ) ) ;
#35493=CARTESIAN_POINT ( 'NONE',  ( 33.79837243370585043, -287.1223522448397034, -287.1832089486352970 ) ) ;
#35494=CARTESIAN_POINT ( 'NONE',  ( -108.1729423791250753, -283.6755887557876008, -300.5384428048024574 ) ) ;
#35495=CARTESIAN_POINT ( 'NONE',  ( -36.98422120466628371, -278.4565726065222862, -196.5619809515205816 ) ) ;
#35496=CARTESIAN_POINT ( 'NONE',  ( -69.32826939448453629, -287.4871641778752291, -203.3566091398639912 ) ) ;
#35497=CARTESIAN_POINT ( 'NONE',  ( 21.07731089913698952, -279.4055687813314535, -225.4192596737672716 ) ) ;
#35498=CARTESIAN_POINT ( 'NONE',  ( 12.09171111390374520, -277.6629190006742647, -324.8138380611150637 ) ) ;
#35499=CARTESIAN_POINT ( 'NONE',  ( 29.21290243875100856, -276.4503908358885838, -300.5020091212221018 ) ) ;
#35500=CARTESIAN_POINT ( 'NONE',  ( -41.75310905305579467, -287.9014657229816407, -346.8500732827675392 ) ) ;
#35501=CARTESIAN_POINT ( 'NONE',  ( -90.31938848510732498, -284.5814777130545394, -326.0894620818544922 ) ) ;
#35502=CARTESIAN_POINT ( 'NONE',  ( -108.9734851424181841, -285.4023364658055470, -242.1374834191706498 ) ) ;
#35503=CARTESIAN_POINT ( 'NONE',  ( 9.274907507419671404, -280.8798851831136290, -214.1178997202809171 ) ) ;
#35505=ORIENTED_EDGE ( 'NONE', *, *, #25991, .T. ) ;
#35507=CARTESIAN_POINT ( 'NONE',  ( 21.46171059445233098, -290.0641252113188671, -318.1566883230302665 ) ) ;
#35508=CARTESIAN_POINT ( 'NONE',  ( -111.1525730702722967, -289.4913092760557447, -250.1805432059843213 ) ) ;
#35509=AXIS2_PLACEMENT_3D ( 'NONE', #72913, #14248, #29834 ) ;
#35510=CARTESIAN_POINT ( 'NONE',  ( -110.5769942451401704, -271.6110516449974739, -270.3491615739666258 ) ) ;
#35511=CARTESIAN_POINT ( 'NONE',  ( 33.31962016774464530, -293.2891678264079474, -300.8318522878861359 ) ) ;
#35512=CARTESIAN_POINT ( 'NONE',  ( -73.90563459685535008, -288.0270258734280446, -334.3583724591348414 ) ) ;
#35513=CARTESIAN_POINT ( 'NONE',  ( 35.05414176113733049, -291.9930243229286475, -285.8106542917220168 ) ) ;
#35515=CARTESIAN_POINT ( 'NONE',  ( 23.84896899855845120, -289.3168631296668423, -310.9159516872866789 ) ) ;
#35516=CARTESIAN_POINT ( 'NONE',  ( 35.77081079830085031, -295.8376638359844719, -253.6410175316879361 ) ) ;
#35517=CARTESIAN_POINT ( 'NONE',  ( 11.14281742901739314, -290.3808272825906442, -327.5821997882495680 ) ) ;
#35518=CARTESIAN_POINT ( 'NONE',  ( -104.3577542164685923, -289.0023027518378171, -236.2041471817235276 ) ) ;
#35519=CARTESIAN_POINT ( 'NONE',  ( -107.7133135273980997, -292.8906291647765556, -244.2741010033949181 ) ) ;
#35520=CARTESIAN_POINT ( 'NONE',  ( -69.10039032661624958, -284.4216962772506463, -336.3658274265531531 ) ) ;
#35521=CARTESIAN_POINT ( 'NONE',  ( 12.05408248477928979, -294.7373705022885702, -213.7035052212461039 ) ) ;
#35523=DIRECTION ( 'NONE',  ( 0.9951408606192332362, 0.000000000000000000, -0.09846150276129254919 ) ) ;
#35524=CARTESIAN_POINT ( 'NONE',  ( -84.79248009415235288, -275.3815228900309080, -211.8219833771299534 ) ) ;
#35526=CARTESIAN_POINT ( 'NONE',  ( -16.09535092101017995, -281.9674356062802758, -340.3696486909981900 ) ) ;
#35527=CARTESIAN_POINT ( 'NONE',  ( -103.5484032776459600, -282.0833372688729810, -305.7091024207979899 ) ) ;
#35528=CARTESIAN_POINT ( 'NONE',  ( -102.9829610885807654, -295.2266793465228147, -310.3033722968134498 ) ) ;
#35529=CARTESIAN_POINT ( 'NONE',  ( 24.65437826159549672, -273.2394950067836703, -229.9326592251921682 ) ) ;
#35530=CARTESIAN_POINT ( 'NONE',  ( -105.6014272423204829, -276.2389187174886729, -300.1875825290283615 ) ) ;
#35531=CARTESIAN_POINT ( 'NONE',  ( -100.3280264514214792, -298.3860290119940828, -232.3943684674912049 ) ) ;
#35532=CARTESIAN_POINT ( 'NONE',  ( -94.38788784590086323, -297.3244233046321483, -316.8686293091461721 ) ) ;
#35534=CARTESIAN_POINT ( 'NONE',  ( -109.2990945701885437, -297.1800825185141548, -283.6492068335287513 ) ) ;
#35536=CARTESIAN_POINT ( 'NONE',  ( 34.37448242459086600, -285.8695467260812393, -293.4954207105848241 ) ) ;
#35537=CARTESIAN_POINT ( 'NONE',  ( -83.18893748377028885, -273.2369908975525163, -213.5541568656866787 ) ) ;
#35538=CARTESIAN_POINT ( 'NONE',  ( 36.67207139781474012, -286.9514167653484265, -249.0127451384059043 ) ) ;
#35539=CARTESIAN_POINT ( 'NONE',  ( -3.934788865591847262, -296.5937064219432386, -337.9208416878618095 ) ) ;
#35540=CARTESIAN_POINT ( 'NONE',  ( 24.10757764472594999, -290.9710883043557601, -227.6300444767181830 ) ) ;
#35542=CARTESIAN_POINT ( 'NONE',  ( -69.88466448665414532, -278.8316166907081879, -200.7399043162345151 ) ) ;
#35544=CARTESIAN_POINT ( 'NONE',  ( -54.42813229853332757, -295.3380690714490129, -195.3538533559490702 ) ) ;
#35546=CARTESIAN_POINT ( 'NONE',  ( -11.86987106776820511, -285.1862079733425048, -201.5256879404417418 ) ) ;
#35548=CARTESIAN_POINT ( 'NONE',  ( 7.007303246093505855, -286.4486423079699762, -330.9086037081987115 ) ) ;
#35549=CARTESIAN_POINT ( 'NONE',  ( 9.546310512083316269, -300.2487942568411086, -196.5480832843507812 ) ) ;
#35550=CARTESIAN_POINT ( 'NONE',  ( -79.60014461081689774, -280.9189174290218034, -206.6357955574420089 ) ) ;
#35551=CARTESIAN_POINT ( 'NONE',  ( -112.4786176582602053, -294.6537535082063641, -263.9840069950697057 ) ) ;
#35552=CARTESIAN_POINT ( 'NONE',  ( -6.032943655893342694, -282.6288903448995029, -336.3200104194942810 ) ) ;
#35553=CARTESIAN_POINT ( 'NONE',  ( -114.3098143371742168, -296.7641514905550935, -266.7373965977121202 ) ) ;
#35554=CARTESIAN_POINT ( 'NONE',  ( -102.5610064780436517, -274.4388730627857171, -236.1652610441418574 ) ) ;
#35555=CARTESIAN_POINT ( 'NONE',  ( -10.48252730804613897, -284.4795664665907111, -199.6803121136453001 ) ) ;
#35556=CARTESIAN_POINT ( 'NONE',  ( -20.23774003576258806, -282.2719182022274254, -197.2841128585155275 ) ) ;
#35557=CARTESIAN_POINT ( 'NONE',  ( -100.0922376137794458, -296.1299664686275719, -232.5030424647576979 ) ) ;
#35560=CARTESIAN_POINT ( 'NONE',  ( -81.58112478838474146, -285.6370029104722335, -330.5479537597688022 ) ) ;
#35562=CARTESIAN_POINT ( 'NONE',  ( -4.829096099716524648, -286.1237833571632905, -337.9475929042657754 ) ) ;
#35563=CARTESIAN_POINT ( 'NONE',  ( 38.57459002123052727, -274.9022556706869977, -282.5638851485002760 ) ) ;
#35564=CARTESIAN_POINT ( 'NONE',  ( -25.40700136800590059, -292.0416943095534066, -198.2918429051778162 ) ) ;
#35565=CARTESIAN_POINT ( 'NONE',  ( 5.308823781287471455, -282.1612441236668474, -210.2641915961094981 ) ) ;
#35566=CARTESIAN_POINT ( 'NONE',  ( 27.47906547556778278, -277.6298989291624935, -305.7484320484457498 ) ) ;
#35567=CARTESIAN_POINT ( 'NONE',  ( 1.701914455523916514, -284.1392592524099996, -335.7983900479193267 ) ) ;
#35568=CARTESIAN_POINT ( 'NONE',  ( 14.19261064637782432, -281.1036916034582873, -322.6949364592601910 ) ) ;
#35569=CARTESIAN_POINT ( 'NONE',  ( -90.91969204759215017, -281.2923472870057822, -217.8051170066295867 ) ) ;
#35570=CARTESIAN_POINT ( 'NONE',  ( -46.12987281963491171, -297.9435993370572078, -193.8642682386428362 ) ) ;
#35571=CARTESIAN_POINT ( 'NONE',  ( 35.20025596961704650, -275.7131136775552136, -296.3381156866676633 ) ) ;
#35572=CARTESIAN_POINT ( 'NONE',  ( 32.16438303110388830, -295.1232582507774964, -243.7111911560612327 ) ) ;
#35573=FACE_OUTER_BOUND ( 'NONE', #25281, .T. ) ;
#35574=CARTESIAN_POINT ( 'NONE',  ( -22.36525510383600590, -293.0019250753132383, -344.6309744000934074 ) ) ;
#35575=CARTESIAN_POINT ( 'NONE',  ( -76.59200930779327621, -273.0188863958001093, -208.7380567888023961 ) ) ;
#35577=CARTESIAN_POINT ( 'NONE',  ( 36.43126210635471551, -295.3186095221691403, -289.8613179153579722 ) ) ;
#35578=CARTESIAN_POINT ( 'NONE',  ( -2.136234668907611489, -295.8015957772047955, -338.3948149389269133 ) ) ;
#35579=CARTESIAN_POINT ( 'NONE',  ( -37.24059935678067745, -291.0510410131372510, -345.1943873888910161 ) ) ;
#35580=CARTESIAN_POINT ( 'NONE',  ( -107.2172423288878207, -276.9026434700369919, -243.4310942860465161 ) ) ;
#35581=CARTESIAN_POINT ( 'NONE',  ( -4.407404038106616184, -278.5349154432033743, -337.1334024252158770 ) ) ;
#35582=CARTESIAN_POINT ( 'NONE',  ( 35.90439305436713369, -291.4592984149966810, -257.0114057549722588 ) ) ;
#35583=CARTESIAN_POINT ( 'NONE',  ( 20.11367479828315652, -282.7348283083477440, -220.9532887883599983 ) ) ;
#35585=CARTESIAN_POINT ( 'NONE',  ( -68.89557852661957327, -284.5475529160565884, -204.1764409460664922 ) ) ;
#35586=CARTESIAN_POINT ( 'NONE',  ( 47.08420963622742050, 10.99842292863093896, -330.8880468998681295 ) ) ;
#35588=CARTESIAN_POINT ( 'NONE',  ( -96.58949594620050050, -284.8158242663156443, -227.6574013950746576 ) ) ;
#35589=CARTESIAN_POINT ( 'NONE',  ( -56.49280826896303864, -280.8907391186834275, -196.0451239601401596 ) ) ;
#35590=CARTESIAN_POINT ( 'NONE',  ( -102.5879497504052580, -282.8197931624920329, -310.4975805594237386 ) ) ;
#35591=CARTESIAN_POINT ( 'NONE',  ( -82.11138006969866865, -280.3991825900214394, -208.0033119734538900 ) ) ;
#35592=CARTESIAN_POINT ( 'NONE',  ( -72.50381948162078061, -279.0290751780003120, -338.0981590714568483 ) ) ;
#35593=CARTESIAN_POINT ( 'NONE',  ( -82.13390479932378696, -299.9090924074130271, -214.2458315076590907 ) ) ;
#35596=CARTESIAN_POINT ( 'NONE',  ( -78.63378679019862716, -299.4966662489894702, -207.6890795956263105 ) ) ;
#35597=CARTESIAN_POINT ( 'NONE',  ( -100.8542679731100975, -277.1022976673459084, -231.0452144819477098 ) ) ;
#35598=CARTESIAN_POINT ( 'NONE',  ( -113.3759036933542603, -292.3011591358191481, -271.2397103727222998 ) ) ;
#35599=CARTESIAN_POINT ( 'NONE',  ( 19.76820487696091888, -293.5446538253959829, -316.0138586652342383 ) ) ;
#35600=CARTESIAN_POINT ( 'NONE',  ( -41.76329274598327856, -288.6140791635320966, -347.1856335842026624 ) ) ;
#35602=CARTESIAN_POINT ( 'NONE',  ( -3.506153775527077521, -293.1890930628226215, -338.8866451305271426 ) ) ;
#35603=CARTESIAN_POINT ( 'NONE',  ( -11.72540053608412869, -284.7912190347873889, -201.1495177252999440 ) ) ;
#35604=CARTESIAN_POINT ( 'NONE',  ( -4.304300342531534262, -294.3526987455283574, -203.8684239043339517 ) ) ;
#35605=CARTESIAN_POINT ( 'NONE',  ( -5.481530360466991603, -284.9588735154609367, -203.8969395708655554 ) ) ;
#35606=CARTESIAN_POINT ( 'NONE',  ( -38.87871202335794152, -284.3869739256532512, -343.8507720152429101 ) ) ;
#35607=CARTESIAN_POINT ( 'NONE',  ( -113.9537707808432856, -291.5540996660268434, -265.5226427393353106 ) ) ;
#35608=CARTESIAN_POINT ( 'NONE',  ( 21.37469264596427720, -281.4351506659519373, -226.8616363258992124 ) ) ;
#35609=CARTESIAN_POINT ( 'NONE',  ( 24.55632620255637022, -292.9494285973721048, -315.5123895803252481 ) ) ;
#35610=CARTESIAN_POINT ( 'NONE',  ( 25.72504150123767985, -288.9372845093539013, -314.3471929137066354 ) ) ;
#35612=CARTESIAN_POINT ( 'NONE',  ( -95.40773584403584096, -290.3616619358701882, -320.8374728391015651 ) ) ;
#35613=CARTESIAN_POINT ( 'NONE',  ( 25.69712109552919088, -288.2252986347052683, -307.2728344847255357 ) ) ;
#35616=CARTESIAN_POINT ( 'NONE',  ( -22.31891828115328025, -296.7221580835962413, -344.6216155800368028 ) ) ;
#35617=CARTESIAN_POINT ( 'NONE',  ( -35.82337579786811688, -296.7556195291638801, -193.8545962127014946 ) ) ;
#35618=CARTESIAN_POINT ( 'NONE',  ( -110.5861044000194511, -277.6434088707502497, -267.8883994169286780 ) ) ;
#35619=CARTESIAN_POINT ( 'NONE',  ( -92.12084595472303761, -272.8025043903053302, -216.3354566199294595 ) ) ;
#35620=CARTESIAN_POINT ( 'NONE',  ( -5.256977876383158055, -293.1019368152330458, -336.7171886361172710 ) ) ;
#35621=CARTESIAN_POINT ( 'NONE',  ( 35.10873661480165708, -277.1146375905308332, -255.1696209777039144 ) ) ;
#35622=CARTESIAN_POINT ( 'NONE',  ( -98.85362310101784544, -271.2608817246718331, -228.7104735480878617 ) ) ;
#35623=CARTESIAN_POINT ( 'NONE',  ( 13.16534093424485619, -293.9825340517983818, -217.1054205664788412 ) ) ;
#35624=CARTESIAN_POINT ( 'NONE',  ( -69.84882497563455672, -296.5703777250566304, -336.0689022153982819 ) ) ;
#35626=CARTESIAN_POINT ( 'NONE',  ( -89.45970809972031645, -293.7836561774128086, -324.5968288064988201 ) ) ;
#35627=CARTESIAN_POINT ( 'NONE',  ( -51.78960768913849932, -298.5235050161888921, -194.7782406503994821 ) ) ;
#35628=CARTESIAN_POINT ( 'NONE',  ( 28.74905534621937164, -286.5617600331370909, -302.7244762176450763 ) ) ;
#35629=CARTESIAN_POINT ( 'NONE',  ( -105.0205097476559644, -274.9777367158422408, -238.0411647941178614 ) ) ;
#35630=CARTESIAN_POINT ( 'NONE',  ( -112.3846526553913776, -273.2569368302204680, -253.3881341676984675 ) ) ;
#35631=CARTESIAN_POINT ( 'NONE',  ( -98.74878486601731709, -296.3376499812720226, -309.9664894402433788 ) ) ;
#35633=CARTESIAN_POINT ( 'NONE',  ( -112.0889811220736050, -280.6592057729443468, -260.4106016565929735 ) ) ;
#35634=CARTESIAN_POINT ( 'NONE',  ( 38.78562209701920693, -280.3392097480020198, -278.4829295093748556 ) ) ;
#35635=CARTESIAN_POINT ( 'NONE',  ( -21.75476477491436711, -282.2059913733568806, -345.6629123341503487 ) ) ;
#35636=CARTESIAN_POINT ( 'NONE',  ( 34.08648801887899538, -275.2642023349746978, -298.9884388004801963 ) ) ;
#35637=CARTESIAN_POINT ( 'NONE',  ( -11.75854859957883924, -278.7795138264719981, -198.5286759895561204 ) ) ;
#35638=CARTESIAN_POINT ( 'NONE',  ( -64.06611331430070777, -277.7043532313207947, -200.0507439231699607 ) ) ;
#35640=CARTESIAN_POINT ( 'NONE',  ( -99.77082865465118289, -271.6603413238086091, -231.3998702102258278 ) ) ;
#35641=CARTESIAN_POINT ( 'NONE',  ( 23.83169745274588180, -276.9623185015346394, -226.9477369890688294 ) ) ;
#35643=CARTESIAN_POINT ( 'NONE',  ( 36.45635138963580602, -291.3766982735485271, -255.0578793968104492 ) ) ;
#35644=CARTESIAN_POINT ( 'NONE',  ( -101.6839608269671089, -291.1092619407325515, -227.9679967971410122 ) ) ;
#35645=CARTESIAN_POINT ( 'NONE',  ( 17.58144542816662792, -278.2692377988443013, -321.6785273975654604 ) ) ;
#35646=CARTESIAN_POINT ( 'NONE',  ( -69.10709424787449962, -271.6342739609892192, -202.4061871036267064 ) ) ;
#35650=CARTESIAN_POINT ( 'NONE',  ( -22.24705103918196514, -284.2451764123570683, -196.8433691840046720 ) ) ;
#35653=CARTESIAN_POINT ( 'NONE',  ( 32.18207957688112941, -292.0342789044797769, -246.6746413627150787 ) ) ;
#35654=CARTESIAN_POINT ( 'NONE',  ( 34.59125077131827197, -285.4530311993144096, -251.9653702247021556 ) ) ;
#35657=CARTESIAN_POINT ( 'NONE',  ( -37.01164480955512204, -293.0478298014481879, -345.3731601704226364 ) ) ;
#35658=CARTESIAN_POINT ( 'NONE',  ( -76.41961876713757817, -282.0442731461977246, -335.9633993510827281 ) ) ;
#35659=CARTESIAN_POINT ( 'NONE',  ( -98.66964972169510872, -280.7173433427058171, -229.2176549231458011 ) ) ;
#35660=CARTESIAN_POINT ( 'NONE',  ( -105.0881373935143870, -286.2225377310180647, -234.4923749928344705 ) ) ;
#35661=CARTESIAN_POINT ( 'NONE',  ( -7.908527205002114258, -278.6723627708439608, -200.2922913497037314 ) ) ;
#35662=CARTESIAN_POINT ( 'NONE',  ( 35.55264398448798602, -287.4891697034146887, -265.5867029780700932 ) ) ;
#35663=CARTESIAN_POINT ( 'NONE',  ( -81.15576975124106696, -279.0861569633106569, -329.4855817737606003 ) ) ;
#35664=CARTESIAN_POINT ( 'NONE',  ( -103.5202686159419443, -279.7769454022767377, -239.0490774802385090 ) ) ;
#35665=CARTESIAN_POINT ( 'NONE',  ( -105.2089308069749478, -286.9613679259056767, -237.6128997148364022 ) ) ;
#35667=CARTESIAN_POINT ( 'NONE',  ( -36.18225594080007568, -297.8996140624144005, -193.3611496608207858 ) ) ;
#35668=CARTESIAN_POINT ( 'NONE',  ( -12.72212176263686523, -290.7104039402578337, -340.8290054400819145 ) ) ;
#35670=CARTESIAN_POINT ( 'NONE',  ( -88.52914483777347243, -281.9090924074130839, -206.2264541496106460 ) ) ;
#35672=CARTESIAN_POINT ( 'NONE',  ( 23.02314523118107203, -272.9419774259030191, -225.5714554022020195 ) ) ;
#35673=CARTESIAN_POINT ( 'NONE',  ( 27.41519983118940118, -292.4839354754254828, -310.6221847946114281 ) ) ;
#35674=CARTESIAN_POINT ( 'NONE',  ( -47.80804525473786981, -294.6963550318693592, -342.7204223099776073 ) ) ;
#35675=CARTESIAN_POINT ( 'NONE',  ( 36.24371113329314653, -289.0090469521384762, -265.5220676799170292 ) ) ;
#35676=CARTESIAN_POINT ( 'NONE',  ( 18.71758528305098679, -282.6332287571396478, -222.0164127441720723 ) ) ;
#35677=CARTESIAN_POINT ( 'NONE',  ( -43.11949770513703584, -290.5490251124095948, -346.5531342840275215 ) ) ;
#35678=CARTESIAN_POINT ( 'NONE',  ( 22.90951944397731310, -289.5017811974460074, -317.5318607374728685 ) ) ;
#35679=CARTESIAN_POINT ( 'NONE',  ( -109.9716663538028314, -286.7926487088613499, -251.6558070265734273 ) ) ;
#35680=CARTESIAN_POINT ( 'NONE',  ( -103.6047097010405054, -278.2067200241035607, -309.6857391723037267 ) ) ;
#35682=CARTESIAN_POINT ( 'NONE',  ( 36.05528065059214526, -291.8614408748849200, -288.3650417386569416 ) ) ;
#35683=CARTESIAN_POINT ( 'NONE',  ( 38.25509172380060363, -281.2024669385270386, -255.7281050929548485 ) ) ;
#35684=CARTESIAN_POINT ( 'NONE',  ( -70.05628937930782740, -275.4768869026192419, -203.7231323141346024 ) ) ;
#35685=CARTESIAN_POINT ( 'NONE',  ( -69.91165696735023971, -288.1233781216987495, -202.8022627189028810 ) ) ;
#35686=CARTESIAN_POINT ( 'NONE',  ( 22.84414049294219140, -273.1645078783168969, -223.9541726910825616 ) ) ;
#35688=CARTESIAN_POINT ( 'NONE',  ( -81.31992600304128871, -278.9437314535050518, -211.9546083853312268 ) ) ;
#35689=CARTESIAN_POINT ( 'NONE',  ( 18.62365015148619207, -277.4742813533255799, -322.6668374275178053 ) ) ;
#35690=CARTESIAN_POINT ( 'NONE',  ( -105.3133474471421067, -298.3525514961377212, -242.1612939324398610 ) ) ;
#35691=CARTESIAN_POINT ( 'NONE',  ( -27.41444184473359513, -281.9878390649325297, -346.5344163940760041 ) ) ;
#35692=CARTESIAN_POINT ( 'NONE',  ( -83.15620781575645992, -291.4496448347164232, -328.4903266148244256 ) ) ;
#35693=CARTESIAN_POINT ( 'NONE',  ( -113.0699119117287950, -274.2592728085912768, -261.8948109620706077 ) ) ;
#35694=CARTESIAN_POINT ( 'NONE',  ( -71.19972443311384325, -274.9296880755725851, -201.7540304111158775 ) ) ;
#35695=CARTESIAN_POINT ( 'NONE',  ( 19.37825820711082869, -296.2306114685429748, -319.1953626746648638 ) ) ;
#35696=CARTESIAN_POINT ( 'NONE',  ( -67.31674705229335132, -281.4459563578201937, -338.9426996510161985 ) ) ;
#35697=CARTESIAN_POINT ( 'NONE',  ( -112.2957123586946722, -290.4382974932345292, -252.8214389033918792 ) ) ;
#35698=CARTESIAN_POINT ( 'NONE',  ( 35.49274659202517768, -273.7838106213210949, -286.7589880351060287 ) ) ;
#35699=CARTESIAN_POINT ( 'NONE',  ( -26.75264705767810725, -287.7846753087542879, -194.8475083008703166 ) ) ;
#35700=CARTESIAN_POINT ( 'NONE',  ( -108.7253268187797204, -289.6924569084037557, -253.6149846006159976 ) ) ;
#35702=CARTESIAN_POINT ( 'NONE',  ( -100.2062359093196875, -288.5488646877317365, -313.7967765379049183 ) ) ;
#35703=CARTESIAN_POINT ( 'NONE',  ( -106.9735466448185690, -289.9254795745940214, -292.5168735078441387 ) ) ;
#35705=CARTESIAN_POINT ( 'NONE',  ( 37.41521308436237803, -288.4162592285081246, -253.1886648918073490 ) ) ;
#35706=CARTESIAN_POINT ( 'NONE',  ( -39.15403469166486872, -277.4088019899522237, -343.3597681775084993 ) ) ;
#35707=CARTESIAN_POINT ( 'NONE',  ( -34.87839844508079068, -293.9422192775799090, -347.0124366629040082 ) ) ;
#35708=CARTESIAN_POINT ( 'NONE',  ( -35.89278673019682486, -283.6858706970404000, -347.2586335577438490 ) ) ;
#35709=CARTESIAN_POINT ( 'NONE',  ( -109.9587174054438634, -285.2077617760877501, -244.8167821481874000 ) ) ;
#35710=CARTESIAN_POINT ( 'NONE',  ( 33.47504669929764987, -281.6498968822420466, -252.5037049940493432 ) ) ;
#35711=CARTESIAN_POINT ( 'NONE',  ( 189.6301554638078244, 271.4469872958309793, -139.6143609917278638 ) ) ;
#35712=CARTESIAN_POINT ( 'NONE',  ( 101.9353623535783981, 116.6993224611678386, -282.1991941425848154 ) ) ;
#35713=CARTESIAN_POINT ( 'NONE',  ( 24.45853180448317588, -23.43590537780826466, -341.6733390498814629 ) ) ;
#35714=CARTESIAN_POINT ( 'NONE',  ( -87.43643810223066737, -272.5290967060798266, -216.9708593713176867 ) ) ;
#35715=CARTESIAN_POINT ( 'NONE',  ( 15.67982577811148026, -273.7446385433290175, -219.6620939320645789 ) ) ;
#35716=CARTESIAN_POINT ( 'NONE',  ( -47.62955460570826460, -294.6872688541436673, -346.6086553418827521 ) ) ;
#35717=CARTESIAN_POINT ( 'NONE',  ( 46.20262913025351992, 10.70065294047900295, -328.7549391094264593 ) ) ;
#35718=CARTESIAN_POINT ( 'NONE',  ( 9.223534236405900089, -273.3616841466711094, -209.6571047707684841 ) ) ;
#35719=CARTESIAN_POINT ( 'NONE',  ( -111.4739401608841121, -298.3618730044814242, -274.2696299215406839 ) ) ;
#35720=CARTESIAN_POINT ( 'NONE',  ( -48.11685016983486918, -290.5071472515609230, -343.1114493814743014 ) ) ;
#35721=CARTESIAN_POINT ( 'NONE',  ( -107.3007046392191199, -291.9214536950478305, -248.4107289403539482 ) ) ;
#35723=CARTESIAN_POINT ( 'NONE',  ( -78.08775392017629713, -298.4597666689002153, -205.3028416987097842 ) ) ;
#35725=CARTESIAN_POINT ( 'NONE',  ( -14.55275688468293360, -286.8478771943365473, -200.8915419411851531 ) ) ;
#35726=CARTESIAN_POINT ( 'NONE',  ( 38.20038889795292647, -294.5320232029475847, -284.4875671691122534 ) ) ;
#35727=CARTESIAN_POINT ( 'NONE',  ( -88.55978787883272219, -296.2399624968351191, -327.8453971409397809 ) ) ;
#35728=CARTESIAN_POINT ( 'NONE',  ( -2.441302814725339942, -292.6941719932141268, -206.2301367280074658 ) ) ;
#35730=CARTESIAN_POINT ( 'NONE',  ( -3.229932089025133291, -276.4191939330307264, -202.9248745331114776 ) ) ;
#35732=CARTESIAN_POINT ( 'NONE',  ( -101.8362077740213891, -278.6123068678450068, -228.3125459905606363 ) ) ;
#35733=CARTESIAN_POINT ( 'NONE',  ( -16.39428891565522761, -272.7271574728490577, -199.5431013742716004 ) ) ;
#35734=CARTESIAN_POINT ( 'NONE',  ( 9.229930784917645070, -299.8529804473018885, -196.9542415464881344 ) ) ;
#35735=CARTESIAN_POINT ( 'NONE',  ( 25.58384586021559670, -277.0068504540777212, -307.8282250205483592 ) ) ;
#35736=CARTESIAN_POINT ( 'NONE',  ( 4.288999983718310816, -276.3648587867934907, -206.7309499166615865 ) ) ;
#35737=CARTESIAN_POINT ( 'NONE',  ( 34.90909198118203705, -273.8472112388758433, -291.8128951153929620 ) ) ;
#35738=CARTESIAN_POINT ( 'NONE',  ( -109.4621264632441040, -297.0462940991317851, -282.2999945447016898 ) ) ;
#35739=CARTESIAN_POINT ( 'NONE',  ( -28.84582845064091927, -293.5172005873548073, -343.5097043233968179 ) ) ;
#35741=CARTESIAN_POINT ( 'NONE',  ( -104.9185423907243830, -278.5681303172277126, -307.1428701550810842 ) ) ;
#35742=CARTESIAN_POINT ( 'NONE',  ( -59.19297676218162962, -277.5096859653685897, -340.0139837811059351 ) ) ;
#35743=CARTESIAN_POINT ( 'NONE',  ( 22.61592798916430525, -285.5967661822577384, -222.8178033497227943 ) ) ;
#35744=CARTESIAN_POINT ( 'NONE',  ( -94.20140499135716539, -299.2332506711222209, -221.1203838538394564 ) ) ;
#35745=CARTESIAN_POINT ( 'NONE',  ( 82.62000873716831961, -301.8234436266066041, -196.4228867002380809 ) ) ;
#35746=CARTESIAN_POINT ( 'NONE',  ( 22.12880004312654236, -286.1540203084305176, -227.6627659026793822 ) ) ;
#35748=CARTESIAN_POINT ( 'NONE',  ( -94.71198856607145444, -277.4448965557360793, -223.5997661955304352 ) ) ;
#35749=CARTESIAN_POINT ( 'NONE',  ( -85.85915613411758329, -277.9390693801459520, -215.0309148531598851 ) ) ;
#35750=CARTESIAN_POINT ( 'NONE',  ( -105.2776397533293817, -286.1332247496409309, -302.2579535769954191 ) ) ;
#35751=CARTESIAN_POINT ( 'NONE',  ( -39.15225920570156859, -278.2804555294076749, -343.7358573806489517 ) ) ;
#35753=CARTESIAN_POINT ( 'NONE',  ( 38.83168960953429405, -273.9265756188825662, -268.3473877790993924 ) ) ;
#35754=CARTESIAN_POINT ( 'NONE',  ( -4.065683449955379558, -275.1544247831729422, -205.2579013259077385 ) ) ;
#35755=CARTESIAN_POINT ( 'NONE',  ( 21.42563208398200914, -282.9092808682374880, -223.4745883359465211 ) ) ;
#35757=CARTESIAN_POINT ( 'NONE',  ( 37.35819362320376769, -289.3263221075469573, -258.9067730182167679 ) ) ;
#35758=CARTESIAN_POINT ( 'NONE',  ( 0.1016626691354874934, -292.5539616869652946, -335.4045937221521285 ) ) ;
#35760=CARTESIAN_POINT ( 'NONE',  ( -16.48477909591456836, -273.0120659692967706, -199.8365492795474552 ) ) ;
#35761=CARTESIAN_POINT ( 'NONE',  ( -27.92659694341521970, -290.3123838423521192, -196.6737761133524316 ) ) ;
#35762=CARTESIAN_POINT ( 'NONE',  ( 198.4603912096053193, 279.4542985770845576, -127.2015713121144529 ) ) ;
#35764=CARTESIAN_POINT ( 'NONE',  ( -67.79511929089275668, -287.9245270392905240, -340.3275171708549465 ) ) ;
#35765=CARTESIAN_POINT ( 'NONE',  ( 6.971419010202898114, -284.8856750332267893, -208.5684967984578009 ) ) ;
#35767=CARTESIAN_POINT ( 'NONE',  ( -2.130893058473325219, -284.0016689284511813, -334.9942056471790579 ) ) ;
#35768=CARTESIAN_POINT ( 'NONE',  ( -103.1534602389561996, -284.9218810746347117, -302.4370002272187321 ) ) ;
#35769=CARTESIAN_POINT ( 'NONE',  ( -104.5488301102956399, -292.9817149725633953, -236.1636130415934929 ) ) ;
#35770=CARTESIAN_POINT ( 'NONE',  ( -95.07343119308772827, -273.5750843044803560, -219.4416568718659164 ) ) ;
#35771=CARTESIAN_POINT ( 'NONE',  ( -97.89017324259570785, -288.0189680198514566, -315.5842550233263637 ) ) ;
#35772=CARTESIAN_POINT ( 'NONE',  ( -35.71150949447974909, -277.0322640413725708, -347.3569829833591598 ) ) ;
#35773=CARTESIAN_POINT ( 'NONE',  ( 36.33339277657601940, -295.3762979524936441, -258.2885446450802078 ) ) ;
#35775=CARTESIAN_POINT ( 'NONE',  ( -106.6662871844225293, -299.4805209788416391, -237.0123917617630980 ) ) ;
#35776=CARTESIAN_POINT ( 'NONE',  ( -95.51701017061657240, -282.6087202723107339, -315.2913177761462293 ) ) ;
#35777=CARTESIAN_POINT ( 'NONE',  ( -87.57258024323981260, -277.3507448689070998, -214.6667795891417825 ) ) ;
#35778=CARTESIAN_POINT ( 'NONE',  ( -3.827864094035249298, -296.8649790477389274, -194.1700559458335817 ) ) ;
#35779=CARTESIAN_POINT ( 'NONE',  ( 33.68359635123288598, -275.1293091870567764, -287.7141103081686424 ) ) ;
#35780=CARTESIAN_POINT ( 'NONE',  ( 35.16186280490963867, -294.8990185131866610, -257.1023748630064460 ) ) ;
#35781=CARTESIAN_POINT ( 'NONE',  ( 35.65993172397911337, -294.5702738797263578, -276.2066457257869843 ) ) ;
#35782=CARTESIAN_POINT ( 'NONE',  ( -8.557931017036427335, -295.9985180532308959, -341.3030176357415826 ) ) ;
#35783=CARTESIAN_POINT ( 'NONE',  ( -94.77475341973931222, -295.7500708638505102, -315.4215706449027721 ) ) ;
#35784=CARTESIAN_POINT ( 'NONE',  ( -90.04898186073360478, -291.7971315190189330, -323.7178710680459517 ) ) ;
#35785=CARTESIAN_POINT ( 'NONE',  ( -67.87940098858975091, -283.6087447183925292, -341.0466810819299326 ) ) ;
#35786=CARTESIAN_POINT ( 'NONE',  ( -5.609662958338034855, -272.6046521313609787, -201.5615300403260903 ) ) ;
#35787=CARTESIAN_POINT ( 'NONE',  ( 38.78589388530826199, -287.2398248088587707, -258.7152248779223100 ) ) ;
#35788=CARTESIAN_POINT ( 'NONE',  ( -77.21355966776269497, -279.5689968616500209, -333.5256334986544857 ) ) ;
#35789=CARTESIAN_POINT ( 'NONE',  ( -57.44751234073129353, -284.8450669311596926, -199.8870005509313330 ) ) ;
#35790=CARTESIAN_POINT ( 'NONE',  ( -94.87370288003533858, -287.8870459161533972, -318.4962138518991424 ) ) ;
#35791=CARTESIAN_POINT ( 'NONE',  ( 197.9737475143014365, 296.4634315385704895, -68.42128063630356394 ) ) ;
#35792=CARTESIAN_POINT ( 'NONE',  ( -17.14885707722984520, -285.8274733178143947, -200.0925741636767157 ) ) ;
#35793=CARTESIAN_POINT ( 'NONE',  ( 36.81131506836469924, -282.9990012263287440, -289.5793139696389744 ) ) ;
#35794=CARTESIAN_POINT ( 'NONE',  ( -96.21833019228341755, -288.9457831250846880, -319.6396334000407364 ) ) ;
#35795=CARTESIAN_POINT ( 'NONE',  ( -112.4514144652794840, -280.3145960139933095, -257.5170053841952722 ) ) ;
#35796=CARTESIAN_POINT ( 'NONE',  ( -111.3461277529025750, -279.6222378719067478, -289.8198421680204433 ) ) ;
#35797=CARTESIAN_POINT ( 'NONE',  ( -74.50396051839560130, -279.3766049704270245, -207.4701722827693118 ) ) ;
#35798=CARTESIAN_POINT ( 'NONE',  ( -70.23804776299030550, -275.5963438220910007, -203.3560650445036799 ) ) ;
#35799=CARTESIAN_POINT ( 'NONE',  ( 33.41656906309316355, -293.9404761935502393, -300.8646278004086412 ) ) ;
#35800=CARTESIAN_POINT ( 'NONE',  ( -69.48867689414198878, -287.4974818992690189, -337.7289047352825264 ) ) ;
#35801=CARTESIAN_POINT ( 'NONE',  ( -19.59309812983185140, -293.8766987957554875, -196.2027023095965887 ) ) ;
#35802=CARTESIAN_POINT ( 'NONE',  ( -109.3466978557941758, -295.6541873522023138, -256.5281938818084768 ) ) ;
#35803=CARTESIAN_POINT ( 'NONE',  ( 18.70485979573221869, -284.1577355837754340, -319.3519061008559561 ) ) ;
#35804=CARTESIAN_POINT ( 'NONE',  ( -108.6134334162905191, -296.0093421270138379, -286.2490857875458232 ) ) ;
#35805=CARTESIAN_POINT ( 'NONE',  ( 19.17851645802307559, -293.9237280147394245, -218.5252459732615478 ) ) ;
#35806=CARTESIAN_POINT ( 'NONE',  ( -9.215783632738521192, -281.0812841903089634, -202.8864894940599584 ) ) ;
#35807=CARTESIAN_POINT ( 'NONE',  ( 37.71786178296748204, -274.4082826995642108, -254.2091094770837572 ) ) ;
#35808=CARTESIAN_POINT ( 'NONE',  ( -3.098661364161939602, -289.2631499489598355, -339.2286659032781699 ) ) ;
#35809=CARTESIAN_POINT ( 'NONE',  ( -109.9314630807485571, -282.4144313842024303, -292.1094843333185054 ) ) ;
#35810=CARTESIAN_POINT ( 'NONE',  ( -112.8464250445575772, -290.6970402503378637, -285.4206052511104303 ) ) ;
#35811=CARTESIAN_POINT ( 'NONE',  ( 31.42073759807091093, -288.2125167344005376, -294.9337581478991979 ) ) ;
#35813=CARTESIAN_POINT ( 'NONE',  ( -72.17143339019004600, -195.1523444700580967, -358.2329797547330372 ) ) ;
#35814=CARTESIAN_POINT ( 'NONE',  ( -12.49039970532447086, -92.45239924107487184, -356.2151309002171615 ) ) ;
#35815=CARTESIAN_POINT ( 'NONE',  ( -85.33152481854864391, -275.1952119285918457, -330.4860931364850671 ) ) ;
#35816=CARTESIAN_POINT ( 'NONE',  ( -98.12206922384847019, -278.3147700226716665, -229.5483537839099029 ) ) ;
#35818=CARTESIAN_POINT ( 'NONE',  ( -2.992133447830128468, -279.4375672508744515, -205.5832059854104727 ) ) ;
#35819=CARTESIAN_POINT ( 'NONE',  ( 34.70345811978169337, -274.8757322465228867, -243.2458185281324177 ) ) ;
#35820=CARTESIAN_POINT ( 'NONE',  ( 204.1738562182569865, 292.3636489450777276, -53.99999999999267430 ) ) ;
#35821=CARTESIAN_POINT ( 'NONE',  ( -74.70385637036221738, -278.1396314869719504, -203.7077191627982984 ) ) ;
#35822=CARTESIAN_POINT ( 'NONE',  ( -97.25671647852421131, -281.9615904925966561, -314.8811990818225013 ) ) ;
#35823=CARTESIAN_POINT ( 'NONE',  ( -104.3704482384691090, -298.7822565502026464, -234.4566871739443457 ) ) ;
#35824=CARTESIAN_POINT ( 'NONE',  ( -85.97466090867335708, -291.8491154946696611, -215.7694116278451588 ) ) ;
#35826=CARTESIAN_POINT ( 'NONE',  ( -100.7377745373110969, -288.7287360421577205, -307.6390872808646009 ) ) ;
#35827=CARTESIAN_POINT ( 'NONE',  ( -46.87659259968729231, -274.5854986846861721, -194.0564745330433425 ) ) ;
#35828=CARTESIAN_POINT ( 'NONE',  ( -109.1297112356303813, -272.7304682825526925, -256.8437820316009947 ) ) ;
#35831=CARTESIAN_POINT ( 'NONE',  ( -47.94142310011969954, -281.8386345904721679, -195.4954448632993547 ) ) ;
#35833=CARTESIAN_POINT ( 'NONE',  ( 33.02746530422345472, -282.3610835660103930, -249.8085845527403421 ) ) ;
#35834=CARTESIAN_POINT ( 'NONE',  ( -50.78269387533965329, -281.6428450905522709, -195.5726583206794089 ) ) ;
#35835=CARTESIAN_POINT ( 'NONE',  ( -108.5916475128085779, -283.8342606845941418, -253.3703990194199775 ) ) ;
#35836=CARTESIAN_POINT ( 'NONE',  ( -109.1737112997808623, -280.6563994718788990, -251.5753916457361186 ) ) ;
#35837=CARTESIAN_POINT ( 'NONE',  ( 35.53014415759140121, -273.8875264506598342, -259.3032789301449839 ) ) ;
#35838=CARTESIAN_POINT ( 'NONE',  ( 145.2857639756989272, -299.5541904835127980, -189.7068768330456123 ) ) ;
#35840=CARTESIAN_POINT ( 'NONE',  ( -112.9049625825611542, -279.1793577268580862, -284.3743818936777075 ) ) ;
#35842=CARTESIAN_POINT ( 'NONE',  ( -84.51696442439769896, -276.2617199649768054, -330.5374356780156404 ) ) ;
#35845=CARTESIAN_POINT ( 'NONE',  ( -110.2764947031228786, -286.2891552171987541, -289.3574583836836496 ) ) ;
#35846=CARTESIAN_POINT ( 'NONE',  ( 28.88903878787332147, -292.3289665526837098, -239.1595139744169956 ) ) ;
#35847=CARTESIAN_POINT ( 'NONE',  ( 23.20206595798455140, -287.5355122723147474, -317.7929195592660108 ) ) ;
#35849=CARTESIAN_POINT ( 'NONE',  ( -30.41442431525060286, -284.3806684431287408, -196.6211690512395762 ) ) ;
#35850=CARTESIAN_POINT ( 'NONE',  ( -109.3000335489130777, -282.9244779913994421, -285.8279545215975759 ) ) ;
#35851=CARTESIAN_POINT ( 'NONE',  ( -94.90636749792419380, -288.1430436631787302, -316.8829739982963929 ) ) ;
#35852=CARTESIAN_POINT ( 'NONE',  ( 35.53594366060141851, -282.8770397174846494, -279.4924914117164008 ) ) ;
#35853=CARTESIAN_POINT ( 'NONE',  ( -52.12579010839287008, -271.8628675853944969, -196.7796558272020491 ) ) ;
#35854=CARTESIAN_POINT ( 'NONE',  ( -105.0824008955871847, -282.4962667108395067, -305.3709732489545559 ) ) ;
#35855=CARTESIAN_POINT ( 'NONE',  ( -109.6566811225870879, -298.2965337832521868, -290.2494103855281082 ) ) ;
#35856=CARTESIAN_POINT ( 'NONE',  ( -109.1664589734814825, -282.8391623287386665, -248.0223609661307762 ) ) ;
#35857=CARTESIAN_POINT ( 'NONE',  ( -99.36801492669393099, -278.9562932844493162, -309.3935241990178611 ) ) ;
#35858=CARTESIAN_POINT ( 'NONE',  ( 36.74542958286263428, -289.3887213943446000, -257.5920177674213392 ) ) ;
#35861=CARTESIAN_POINT ( 'NONE',  ( 12.46534283833557666, -296.2852212115566317, -327.2510415009658686 ) ) ;
#35862=CARTESIAN_POINT ( 'NONE',  ( -110.1188386758993261, -276.3185844338349284, -288.5383938779753521 ) ) ;
#35863=CARTESIAN_POINT ( 'NONE',  ( -106.3729476996660566, -289.3137027838367317, -304.2288814774816501 ) ) ;
#35864=CARTESIAN_POINT ( 'NONE',  ( 14.86799095559641870, -292.7014616147563402, -322.5922116243596633 ) ) ;
#35865=CARTESIAN_POINT ( 'NONE',  ( 0.6692559086183191841, -279.2548770556284126, -207.4021954739244507 ) ) ;
#35866=CARTESIAN_POINT ( 'NONE',  ( -88.30162822418512292, -271.4119551560722812, -216.0282409862622046 ) ) ;
#35867=CARTESIAN_POINT ( 'NONE',  ( -30.77950644801808977, -293.4520169201267095, -197.1615203598858841 ) ) ;
#35868=CARTESIAN_POINT ( 'NONE',  ( -54.42813229853332757, -279.7662352645559736, -345.3683826091709648 ) ) ;
#35869=CARTESIAN_POINT ( 'NONE',  ( 1.400589923602379328, -293.0241885309461622, -336.1010808217097292 ) ) ;
#35870=CARTESIAN_POINT ( 'NONE',  ( -100.9836276131071600, -291.6435689623929193, -307.8267549743551399 ) ) ;
#35871=CARTESIAN_POINT ( 'NONE',  ( 25.66538900130607459, -291.2238618999442679, -227.7940489043524224 ) ) ;
#35873=CARTESIAN_POINT ( 'NONE',  ( -71.42970933976185677, -290.9368117308164869, -335.5933148208285957 ) ) ;
#35875=CARTESIAN_POINT ( 'NONE',  ( -73.61616102243436899, -290.3496054595977967, -333.9111032647531943 ) ) ;
#35876=DIRECTION ( 'NONE',  ( 0.000000000000000000, 0.000000000000000000, -1.000000000000000000 ) ) ;
#35877=CARTESIAN_POINT ( 'NONE',  ( -81.71293537649171412, -292.6676974693359625, -207.9175258363220564 ) ) ;
#35878=CARTESIAN_POINT ( 'NONE',  ( 21.60479574164332561, -278.9298727412668768, -223.3968255557733755 ) ) ;
#35879=CARTESIAN_POINT ( 'NONE',  ( -81.72904545615023153, -291.4286961341201732, -212.3423116172144489 ) ) ;
#35880=CARTESIAN_POINT ( 'NONE',  ( -95.89248886396806881, -279.5598684884321301, -220.3653823007524863 ) ) ;
#35881=CARTESIAN_POINT ( 'NONE',  ( 33.15528250359770368, -280.8244693569112087, -239.4431663804909647 ) ) ;
#35882=CARTESIAN_POINT ( 'NONE',  ( 21.93665262005682237, -284.9221397388207038, -224.4146540452813667 ) ) ;
#35884=CARTESIAN_POINT ( 'NONE',  ( 19.42382688510289768, -280.3602386447441290, -318.2195343636670941 ) ) ;
#35885=CARTESIAN_POINT ( 'NONE',  ( -37.94024538081043119, -284.0444955579608290, -195.3635020417542307 ) ) ;
#35887=CARTESIAN_POINT ( 'NONE',  ( -96.52899969924932577, -276.3797080960275707, -318.5435135066287557 ) ) ;
#35888=CARTESIAN_POINT ( 'NONE',  ( -99.42289277995428165, -273.8880870927927731, -231.6503023657550386 ) ) ;
#35890=CARTESIAN_POINT ( 'NONE',  ( -101.8325759346736419, -292.6387921538587875, -234.3762031830789851 ) ) ;
#35891=CARTESIAN_POINT ( 'NONE',  ( -24.27833677943826274, -275.6409346657578681, -195.0215473671578366 ) ) ;
#35892=CARTESIAN_POINT ( 'NONE',  ( -7.502893733694051548, -276.3165191749701535, -337.0074466121967021 ) ) ;
#35893=CARTESIAN_POINT ( 'NONE',  ( 0.2664088270362876543, -296.5518716179108765, -335.3097752432576613 ) ) ;
#35894=CARTESIAN_POINT ( 'NONE',  ( -43.18017833146507201, -289.2906359675313297, -347.1394494099674830 ) ) ;
#35895=CARTESIAN_POINT ( 'NONE',  ( 20.87712562472719569, -278.9722352924721918, -222.1959591063992434 ) ) ;
#35896=CARTESIAN_POINT ( 'NONE',  ( -42.05184177742446394, -291.8276416329142080, -193.5053142319234780 ) ) ;
#35897=CARTESIAN_POINT ( 'NONE',  ( -109.9316994606314637, -289.7433907783371865, -260.2849011877294743 ) ) ;
#35898=CARTESIAN_POINT ( 'NONE',  ( -2.908968490600246870, -292.5968778742449672, -336.9898478507655000 ) ) ;
#35901=CARTESIAN_POINT ( 'NONE',  ( 2.279133542742972640, -292.1059960429151943, -208.9156975273704404 ) ) ;
#35903=CARTESIAN_POINT ( 'NONE',  ( -67.68488546085839630, -271.1237833571632905, -207.2794874003663779 ) ) ;
#35904=CARTESIAN_POINT ( 'NONE',  ( -92.53618087868541409, -294.8778100336870693, -323.7126831653220052 ) ) ;
#35905=CARTESIAN_POINT ( 'NONE',  ( -98.95710847973568036, -286.4747001422683752, -224.9215309864172241 ) ) ;
#35906=CARTESIAN_POINT ( 'NONE',  ( 34.56777083021366792, -287.2158780779911353, -257.5050147388474784 ) ) ;
#35907=CARTESIAN_POINT ( 'NONE',  ( 35.79665274808300524, -277.1955717858698449, -279.7960810334030270 ) ) ;
#35908=CARTESIAN_POINT ( 'NONE',  ( 9.235256765963400838, -292.4293254916535147, -328.7579145080817966 ) ) ;
#35909=CARTESIAN_POINT ( 'NONE',  ( 35.06351440005865072, -295.5127370837394096, -285.7666654754575006 ) ) ;
#35910=CARTESIAN_POINT ( 'NONE',  ( -37.82770890019034482, -275.8532590699784919, -343.7691034773999377 ) ) ;
#35913=CARTESIAN_POINT ( 'NONE',  ( -113.3679943625155175, -296.3709421736039076, -258.2050748188232774 ) ) ;
#35914=CARTESIAN_POINT ( 'NONE',  ( -39.98504682171709845, -291.0056509608852480, -344.8047284580619589 ) ) ;
#35916=CARTESIAN_POINT ( 'NONE',  ( -37.26774325382954345, -299.1327251845659134, -193.6694534736314779 ) ) ;
#35917=CARTESIAN_POINT ( 'NONE',  ( 23.61448049025223028, -287.6433958573451832, -229.9180713994797145 ) ) ;
#35919=CARTESIAN_POINT ( 'NONE',  ( 15.00966031843823245, -279.8275142907165218, -214.1443839329539003 ) ) ;
#35920=CARTESIAN_POINT ( 'NONE',  ( -74.54975851904841022, -296.1848026193763985, -337.7176519130306360 ) ) ;
#35921=CARTESIAN_POINT ( 'NONE',  ( -36.13073356646869172, -287.1767450163325179, -346.1291438599660069 ) ) ;
#35922=CARTESIAN_POINT ( 'NONE',  ( -69.51521488416017291, -295.7973987926621930, -340.3084376610596564 ) ) ;
#35923=CARTESIAN_POINT ( 'NONE',  ( 22.60286574353643729, -293.3041532455619631, -228.6409289324111285 ) ) ;
#35927=CARTESIAN_POINT ( 'NONE',  ( 36.83505127818909131, -289.2988652670415490, -288.3193737197967152 ) ) ;
#35928=CARTESIAN_POINT ( 'NONE',  ( -88.52914483777347243, -287.1952119285918457, -334.4957818155094174 ) ) ;
#35929=CARTESIAN_POINT ( 'NONE',  ( -77.43228425001780124, -278.8782056059986871, -204.6789177783452089 ) ) ;
#35930=CARTESIAN_POINT ( 'NONE',  ( -5.223540613919172237, -284.6287268044742405, -337.9655420994542965 ) ) ;
#35931=CARTESIAN_POINT ( 'NONE',  ( -113.5626383055736426, -283.2035593823263753, -264.2769435574415979 ) ) ;
#35932=CARTESIAN_POINT ( 'NONE',  ( 32.74716778369376158, -285.9594446539716159, -295.4382946877983045 ) ) ;
#35933=CARTESIAN_POINT ( 'NONE',  ( 38.38990711771787545, -277.4583277372731231, -273.9612593269754370 ) ) ;
#35934=CARTESIAN_POINT ( 'NONE',  ( -29.99195762371079610, -274.4810204064551158, -197.7107995257357516 ) ) ;
#35935=ORIENTED_EDGE ( 'NONE', *, *, #46451, .T. ) ;
#35936=CARTESIAN_POINT ( 'NONE',  ( -41.08095014715326698, -293.7849822740155901, -343.7717365995626437 ) ) ;
#35937=CARTESIAN_POINT ( 'NONE',  ( -107.8202617599682611, -278.3009134815028460, -289.3814321308679496 ) ) ;
#35938=CARTESIAN_POINT ( 'NONE',  ( -110.2706850432613237, -277.8254170273582986, -276.0786069709569119 ) ) ;
#35939=CARTESIAN_POINT ( 'NONE',  ( 37.33076981444173725, -276.4116857576322559, -252.8250571644439901 ) ) ;
#35940=CARTESIAN_POINT ( 'NONE',  ( -112.8425207458116830, -277.5098449731387404, -257.4137319488613116 ) ) ;
#35941=CARTESIAN_POINT ( 'NONE',  ( -57.32492746522063243, -168.5919582920984965, -361.8708629427547407 ) ) ;
#35943=CARTESIAN_POINT ( 'NONE',  ( -109.3021001887156416, -298.3042791699436407, -244.6646762997305018 ) ) ;
#35944=CARTESIAN_POINT ( 'NONE',  ( -20.19161114001083490, -279.3376638359844719, -345.3538533559490702 ) ) ;
#35946=CARTESIAN_POINT ( 'NONE',  ( 82.64534425881677748, -299.8335964094648034, -192.8708706794661509 ) ) ;
#35947=CARTESIAN_POINT ( 'NONE',  ( -91.75987617780724293, -286.3330092501024637, -221.1653526072449552 ) ) ;
#35948=CARTESIAN_POINT ( 'NONE',  ( -18.45584352790105243, -288.0522069390998467, -196.7044456223308089 ) ) ;
#35949=CARTESIAN_POINT ( 'NONE',  ( 35.55285048385430002, -286.9815796920115645, -276.4981385649771823 ) ) ;
#35950=CARTESIAN_POINT ( 'NONE',  ( -97.52833812884441045, -284.7020046198523460, -222.4330937194190483 ) ) ;
#35951=CARTESIAN_POINT ( 'NONE',  ( 27.16790575827264931, -279.4672489902299048, -234.5149025364347040 ) ) ;
#35952=CARTESIAN_POINT ( 'NONE',  ( 17.79237646302278364, -288.7123910101200863, -220.6319972394503850 ) ) ;
#35953=CARTESIAN_POINT ( 'NONE',  ( -7.702995656680331926, -278.9276765446437025, -202.8769132350293205 ) ) ;
#35954=CARTESIAN_POINT ( 'NONE',  ( -66.98632753178294763, -278.7642342872966310, -337.6102038145389201 ) ) ;
#35955=CARTESIAN_POINT ( 'NONE',  ( 34.18029930946099881, -275.8470486854521369, -255.3805479684553745 ) ) ;
#35956=CARTESIAN_POINT ( 'NONE',  ( 20.26411540205024764, -287.0339640099466010, -320.8742275618199074 ) ) ;
#35957=CARTESIAN_POINT ( 'NONE',  ( -50.05669831860699759, -284.0131449892352293, -346.1940824747232455 ) ) ;
#35958=CARTESIAN_POINT ( 'NONE',  ( 26.67416482063226724, -282.6067064476460473, -313.0401050614949554 ) ) ;
#35962=CARTESIAN_POINT ( 'NONE',  ( -37.47524285369376429, -290.9141804616032232, -346.1386665567623595 ) ) ;
#35963=CARTESIAN_POINT ( 'NONE',  ( -113.3258391799145954, -289.1190904959850059, -279.7271718684771145 ) ) ;
#35964=CARTESIAN_POINT ( 'NONE',  ( -96.46424865163734808, -272.2151832899973556, -227.0572939716278995 ) ) ;
#35965=CARTESIAN_POINT ( 'NONE',  ( 34.37077811291285911, -292.5469449500603787, -242.4536423903509501 ) ) ;
#35966=CARTESIAN_POINT ( 'NONE',  ( -110.4799782128428092, -288.9140540002245530, -279.3888547370207220 ) ) ;
#35967=CARTESIAN_POINT ( 'NONE',  ( 31.78268359051463676, -291.4435557515766391, -243.9075059910906305 ) ) ;
#35968=CARTESIAN_POINT ( 'NONE',  ( 23.08548225642544338, -289.3345534916576298, -312.0448444051788783 ) ) ;
#35969=CARTESIAN_POINT ( 'NONE',  ( -4.771743288812468897, -297.1233781216987495, -337.9199732462171255 ) ) ;
#35970=CARTESIAN_POINT ( 'NONE',  ( 15.30079172572841983, -290.3092396135111812, -323.8540385873101854 ) ) ;
#35971=CARTESIAN_POINT ( 'NONE',  ( -50.22644223858247869, -289.8878837468391225, -196.3070036835548819 ) ) ;
#35972=CARTESIAN_POINT ( 'NONE',  ( 2.113205009760168451, -294.5801435537571251, -206.5176132412560719 ) ) ;
#35973=CARTESIAN_POINT ( 'NONE',  ( -107.2067417246463066, -285.2032612896694559, -292.3220927090198415 ) ) ;
#35974=CARTESIAN_POINT ( 'NONE',  ( -17.14431014670264375, -294.3124661091924281, -197.9588123442455867 ) ) ;
#35977=CARTESIAN_POINT ( 'NONE',  ( -112.2309057073502743, -274.6389754008060891, -261.9936996624375638 ) ) ;
#35978=CARTESIAN_POINT ( 'NONE',  ( 35.86426593198129353, -280.7620156665488480, -271.3260681264384857 ) ) ;
#35979=CARTESIAN_POINT ( 'NONE',  ( -100.7347939852731145, -282.0118106665311757, -310.5372700994254842 ) ) ;
#35980=CARTESIAN_POINT ( 'NONE',  ( -69.46973829306152481, -294.6614688339735721, -340.1748627454306870 ) ) ;
#35981=CARTESIAN_POINT ( 'NONE',  ( -16.33184127520627271, -272.5671703946092066, -199.3389479500310983 ) ) ;
#35982=CARTESIAN_POINT ( 'NONE',  ( -86.06589630116212675, -275.8131726462228244, -326.7078955979637840 ) ) ;
#35983=CARTESIAN_POINT ( 'NONE',  ( -107.9377117754009134, -298.1357512147263833, -249.9296075600573772 ) ) ;
#35984=CARTESIAN_POINT ( 'NONE',  ( -5.268421674030641100, -296.0468539821069385, -336.6070564659072488 ) ) ;
#35986=CARTESIAN_POINT ( 'NONE',  ( 14.43777369014532930, -295.1040353204406870, -322.1187978897140738 ) ) ;
#35988=CARTESIAN_POINT ( 'NONE',  ( -0.4979073383079692383, -284.5593644069957122, -204.6125189248627976 ) ) ;
#35989=CARTESIAN_POINT ( 'NONE',  ( -100.1664722097354172, -296.0401386917951072, -307.6365571505736511 ) ) ;
#35990=CARTESIAN_POINT ( 'NONE',  ( -93.43153693400074644, -283.8319477712225876, -323.1339330929971538 ) ) ;
#35991=AXIS2_PLACEMENT_3D ( 'NONE', #16573, #59692, #74328 ) ;
#35992=CARTESIAN_POINT ( 'NONE',  ( 35.83026231740477385, -286.9160724351013414, -246.2822878044025003 ) ) ;
#35993=CARTESIAN_POINT ( 'NONE',  ( -61.04964880909157898, -297.3381486891323675, -341.9442544535156685 ) ) ;
#35994=CARTESIAN_POINT ( 'NONE',  ( 23.30507938420539915, -290.9534921414048085, -226.4987368238243448 ) ) ;
#35995=CARTESIAN_POINT ( 'NONE',  ( -107.2679199732858990, -278.1587454728679631, -238.3821078083812495 ) ) ;
#35996=CARTESIAN_POINT ( 'NONE',  ( 31.95455697924147387, -285.4809262143061801, -303.7686719486574134 ) ) ;
#35997=DIRECTION ( 'NONE',  ( -1.000000000000000000, -0.000000000000000000, -0.000000000000000000 ) ) ;
#35998=CARTESIAN_POINT ( 'NONE',  ( 0.3858672293007937570, -285.3614245582684248, -207.3434506458920623 ) ) ;
#36002=CARTESIAN_POINT ( 'NONE',  ( -108.7384034567929518, -297.9077319520077936, -289.0912630905892797 ) ) ;
#36003=CARTESIAN_POINT ( 'NONE',  ( -33.95965310423532202, -281.5191842455809592, -194.0252283119619392 ) ) ;
#36004=CARTESIAN_POINT ( 'NONE',  ( -99.38186327574641155, -295.1495617136193914, -227.5666745904416928 ) ) ;
#36005=CARTESIAN_POINT ( 'NONE',  ( -16.13250130004695748, -282.7701389099767653, -340.2121729858519075 ) ) ;
#36006=CARTESIAN_POINT ( 'NONE',  ( -113.1394902320587619, -296.8883355883930335, -256.8077043951365113 ) ) ;
#36007=CARTESIAN_POINT ( 'NONE',  ( -63.34203998585009998, -299.2274142097465983, -201.3528631349783211 ) ) ;
#36008=CARTESIAN_POINT ( 'NONE',  ( 36.88036766833413083, -285.4515845579388724, -256.2048878173302455 ) ) ;
#36010=CARTESIAN_POINT ( 'NONE',  ( -109.4223383124809317, -280.8190351025744462, -249.6395772778710977 ) ) ;
#36011=CARTESIAN_POINT ( 'NONE',  ( -65.65264073796910793, -296.7313028557964572, -202.8192858317003981 ) ) ;
#36014=CARTESIAN_POINT ( 'NONE',  ( -90.03799071820556321, -285.7805930399254635, -323.3009071382941784 ) ) ;
#36016=CARTESIAN_POINT ( 'NONE',  ( -85.28047601435909542, -282.9094976428775681, -210.1954327657594206 ) ) ;
#36017=CARTESIAN_POINT ( 'NONE',  ( 29.81139469213858817, -274.2629953692501203, -232.9070604222078202 ) ) ;
#36018=CARTESIAN_POINT ( 'NONE',  ( 30.82914868770197714, -293.0367602763806190, -244.2510552437138927 ) ) ;
#36019=CARTESIAN_POINT ( 'NONE',  ( 35.71755542012938633, -282.9412769274255197, -260.3360734027672265 ) ) ;
#36021=CARTESIAN_POINT ( 'NONE',  ( 14.30559291453952220, -277.9119945697760841, -323.1485080595585941 ) ) ;
#36022=CARTESIAN_POINT ( 'NONE',  ( -49.94095544460658687, -284.8103124484644013, -345.5656071417282078 ) ) ;
#36023=CARTESIAN_POINT ( 'NONE',  ( 25.89337390959351026, -280.8573242301625328, -307.7235039038418449 ) ) ;
#36024=CARTESIAN_POINT ( 'NONE',  ( -103.9433420287878107, -281.0100932150013477, -235.7629195286055790 ) ) ;
#36025=CARTESIAN_POINT ( 'NONE',  ( -76.43455178122212601, -273.7114879240963319, -203.9613669617654068 ) ) ;
#36026=CARTESIAN_POINT ( 'NONE',  ( 37.28575135553037256, -275.1481372145277078, -251.3942128689417643 ) ) ;
#36027=CARTESIAN_POINT ( 'NONE',  ( 34.00229101283765232, -295.1945003886354471, -248.9387161770248156 ) ) ;
#36030=CARTESIAN_POINT ( 'NONE',  ( 24.68951602234481868, -292.2766482646951545, -313.8858616748576651 ) ) ;
#36032=CARTESIAN_POINT ( 'NONE',  ( 11.59238728939789986, -274.2605113655901050, -216.0394790837535766 ) ) ;
#36033=CARTESIAN_POINT ( 'NONE',  ( -25.15144851101744194, -293.7250088159098027, -195.0344592441111047 ) ) ;
#36034=CARTESIAN_POINT ( 'NONE',  ( 21.31550574532285580, -284.6948066931273615, -317.0979686699210447 ) ) ;
#36035=CARTESIAN_POINT ( 'NONE',  ( -11.30273312026978516, -293.5889631587131703, -198.2638520161769407 ) ) ;
#36036=CARTESIAN_POINT ( 'NONE',  ( -76.81469423215196457, -291.5822160145771136, -333.9371446128778871 ) ) ;
#36037=CARTESIAN_POINT ( 'NONE',  ( -108.9748653721970157, -276.8316147081663985, -248.7112204203098997 ) ) ;
#36038=CARTESIAN_POINT ( 'NONE',  ( -93.80320085285353571, -279.7949379966387937, -318.8731075945761404 ) ) ;
#36039=CARTESIAN_POINT ( 'NONE',  ( -28.75365586934023554, -293.0223985715033450, -344.3560854813433707 ) ) ;
#36040=CARTESIAN_POINT ( 'NONE',  ( 38.47427313575620644, -283.4068803728491730, -269.9135330446234207 ) ) ;
#36041=CARTESIAN_POINT ( 'NONE',  ( -13.44152678679741086, -281.6548426100673055, -339.7186813489938118 ) ) ;
#36043=CARTESIAN_POINT ( 'NONE',  ( 9.919151263593899870, -282.0469650887955595, -326.0917758862202618 ) ) ;
#36044=CARTESIAN_POINT ( 'NONE',  ( -38.18037391631578714, -281.1215382646490752, -193.6748145284742009 ) ) ;
#36045=CARTESIAN_POINT ( 'NONE',  ( -110.3120082757571794, -283.0520183596102015, -293.7141185224048172 ) ) ;
#36046=CARTESIAN_POINT ( 'NONE',  ( -112.2521607238216035, -279.2830203613024764, -287.1314223183925378 ) ) ;
#36047=CARTESIAN_POINT ( 'NONE',  ( -82.12360743858742751, -279.1708348516762612, -332.1453273622139477 ) ) ;
#36048=CARTESIAN_POINT ( 'NONE',  ( -105.5795714935544112, -298.8376638359844719, -285.9686137636504668 ) ) ;
#36051=CARTESIAN_POINT ( 'NONE',  ( -89.53538278272077378, -299.3172587367963615, -216.4293233262237663 ) ) ;
#36052=CARTESIAN_POINT ( 'NONE',  ( -94.88986917784711750, -275.9130159801692344, -317.9211897202442287 ) ) ;
#36053=CARTESIAN_POINT ( 'NONE',  ( -58.67593673882629446, -293.5400804007318811, -197.4308474503789057 ) ) ;
#36054=CARTESIAN_POINT ( 'NONE',  ( 35.72347447959032962, -292.8701997590976589, -268.0431603906367855 ) ) ;
#36055=CARTESIAN_POINT ( 'NONE',  ( -34.67523727084896734, -288.5271409076464693, -347.2533599789834398 ) ) ;
#36057=CARTESIAN_POINT ( 'NONE',  ( 22.69733833132485756, -292.7640681905851352, -317.6464692267282430 ) ) ;
#36058=CARTESIAN_POINT ( 'NONE',  ( 7.428238399418281901, -285.0737673624904573, -211.6271832805844610 ) ) ;
#36059=CARTESIAN_POINT ( 'NONE',  ( -95.26940642525214287, -293.0579227246906839, -223.9162803048484989 ) ) ;
#36060=CARTESIAN_POINT ( 'NONE',  ( -39.97953290717646979, -284.4982838564886833, -196.7150074804497990 ) ) ;
#36061=CARTESIAN_POINT ( 'NONE',  ( 21.41418920589967456, -283.4832875887590831, -314.5292747608009449 ) ) ;
#36062=CARTESIAN_POINT ( 'NONE',  ( -38.90333493461796621, -290.0125429811660638, -347.1099388892132538 ) ) ;
#36063=CARTESIAN_POINT ( 'NONE',  ( -24.87204739732126058, -280.7078826319194604, -198.3715617798361563 ) ) ;
#36064=CARTESIAN_POINT ( 'NONE',  ( 29.22199726182032364, -292.8431909825834509, -308.3797495876948460 ) ) ;
#36065=CARTESIAN_POINT ( 'NONE',  ( -6.974314153894478174, -289.4665338820295233, -340.9584765960046866 ) ) ;
#36066=CARTESIAN_POINT ( 'NONE',  ( -65.41871858278739182, -289.9017306944202232, -342.0498639999348143 ) ) ;
#36067=CARTESIAN_POINT ( 'NONE',  ( -105.5656866611570024, -285.0655859301717214, -244.3902176126077563 ) ) ;
#36070=CARTESIAN_POINT ( 'NONE',  ( -14.13745576728970477, -296.6147329282335932, -342.4850981996587507 ) ) ;
#36071=CARTESIAN_POINT ( 'NONE',  ( -81.60015338384043559, -294.3251199883722506, -332.8316626668808453 ) ) ;
#36072=CARTESIAN_POINT ( 'NONE',  ( -98.18241759816103809, -278.1763729420327422, -229.5057189560954782 ) ) ;
#36073=CARTESIAN_POINT ( 'NONE',  ( -101.1539947238558455, -272.6276161224485008, -227.2835178636804585 ) ) ;
#36074=CARTESIAN_POINT ( 'NONE',  ( -82.80259452368517259, -294.1662509362652713, -328.4263195235254784 ) ) ;
#36075=CARTESIAN_POINT ( 'NONE',  ( 30.08654156860731632, -277.7179808264780263, -300.8800667299840370 ) ) ;
#36076=CARTESIAN_POINT ( 'NONE',  ( -92.92759666765854831, -271.3830875816646540, -221.1567118011929267 ) ) ;
#36077=CARTESIAN_POINT ( 'NONE',  ( 14.60811261049018306, -295.5062136478746879, -322.2818715579534796 ) ) ;
#36078=CARTESIAN_POINT ( 'NONE',  ( -103.0390978787870750, -297.1913692566685654, -303.0039009459678141 ) ) ;
#36080=CARTESIAN_POINT ( 'NONE',  ( -95.11896568555668807, -293.8893466703573836, -318.4624883155148609 ) ) ;
#36081=CARTESIAN_POINT ( 'NONE',  ( -35.48331144383948299, -298.7262563450054813, -193.4628507519142033 ) ) ;
#36082=CARTESIAN_POINT ( 'NONE',  ( -82.28943665980462185, -275.4394140254975127, -210.2567668775636776 ) ) ;
#36083=CARTESIAN_POINT ( 'NONE',  ( -107.1728276478716424, -291.1998071498833838, -292.5973368350095143 ) ) ;
#36084=CARTESIAN_POINT ( 'NONE',  ( -5.528460655804314783, -294.9550397425869619, -336.1016801320116656 ) ) ;
#36085=CARTESIAN_POINT ( 'NONE',  ( -104.8601920155234097, -280.0912315486333455, -303.9397612074504877 ) ) ;
#36086=CARTESIAN_POINT ( 'NONE',  ( -79.62419890423167601, -278.1789125132446543, -206.5363926290765164 ) ) ;
#36087=CARTESIAN_POINT ( 'NONE',  ( -37.32261616562219331, -282.4004734249032822, -347.2722309324539083 ) ) ;
#36088=CARTESIAN_POINT ( 'NONE',  ( 38.63372606223966699, -275.0536505971246015, -282.5714272009927299 ) ) ;
#36089=CARTESIAN_POINT ( 'NONE',  ( -98.77073766801068189, -277.5573952300843530, -225.2512589974267314 ) ) ;
#36090=CARTESIAN_POINT ( 'NONE',  ( -1.974970567337443805, -278.5192938369738727, -204.0344802787012100 ) ) ;
#36091=CARTESIAN_POINT ( 'NONE',  ( -107.7550556810145110, -271.4098443262947171, -248.8013328842553449 ) ) ;
#36092=CARTESIAN_POINT ( 'NONE',  ( 14.83968657196227170, -278.3174682628719552, -324.3036662464737105 ) ) ;
#36095=CARTESIAN_POINT ( 'NONE',  ( 35.83096562836566790, -291.3421151222876233, -252.3564576761066007 ) ) ;
#36096=CARTESIAN_POINT ( 'NONE',  ( -104.6099768869517987, -291.0379081191270529, -232.8914109928861649 ) ) ;
#36097=CARTESIAN_POINT ( 'NONE',  ( 22.16545967015004592, -276.9242011598900035, -224.4171277122600543 ) ) ;
#36098=CARTESIAN_POINT ( 'NONE',  ( -112.3407520386660252, -270.5882458039783387, -267.5372233972520917 ) ) ;
#36099=CARTESIAN_POINT ( 'NONE',  ( -67.11703004482465929, -284.8687720866598738, -199.5261792228695867 ) ) ;
#36101=CARTESIAN_POINT ( 'NONE',  ( -111.2706959294984443, -282.7151187825085685, -257.6564226164061324 ) ) ;
#36104=CARTESIAN_POINT ( 'NONE',  ( 33.01409034714732371, -292.0697750463023112, -249.2766881751722110 ) ) ;
#36105=CARTESIAN_POINT ( 'NONE',  ( -72.94596188093042599, -283.7147452805493799, -205.2067978766801275 ) ) ;
#36108=CARTESIAN_POINT ( 'NONE',  ( 34.55341498742018302, -291.2748186305441891, -248.8256107140244069 ) ) ;
#36109=CARTESIAN_POINT ( 'NONE',  ( -103.8225608363302968, -282.5403751060389936, -307.9248652838684848 ) ) ;
#36110=CARTESIAN_POINT ( 'NONE',  ( -109.5432677627753861, -279.9529435662199148, -285.6377029558079812 ) ) ;
#36111=CARTESIAN_POINT ( 'NONE',  ( -111.8294181819885580, -285.5317876106329891, -288.2936401661785908 ) ) ;
#36112=CARTESIAN_POINT ( 'NONE',  ( 0.1686625972033692078, -286.5663059486057591, -207.6765310297049894 ) ) ;
#36114=CARTESIAN_POINT ( 'NONE',  ( -103.6541636890630684, -279.5477988865100087, -302.3855822783746703 ) ) ;
#36115=CARTESIAN_POINT ( 'NONE',  ( -104.4153484784346375, -278.9614671629792042, -299.7066355650611627 ) ) ;
#36116=CARTESIAN_POINT ( 'NONE',  ( -13.25386239782711151, -288.3433976551850719, -198.9595572518784934 ) ) ;
#36118=CARTESIAN_POINT ( 'NONE',  ( -43.28763838203731495, -297.8124832326483897, -193.5378236265038652 ) ) ;
#36119=CARTESIAN_POINT ( 'NONE',  ( 9.020825600810162825, -290.3921225341840113, -328.8620838514359548 ) ) ;
#36120=DIRECTION ( 'NONE',  ( -1.000000000000000000, -0.000000000000000000, -0.000000000000000000 ) ) ;
#36121=CARTESIAN_POINT ( 'NONE',  ( -55.63300648810263738, -282.3376638359844151, -190.3683826091709363 ) ) ;
#36123=CARTESIAN_POINT ( 'NONE',  ( 38.64485042180249508, -291.8799963969167948, -264.6615961247072732 ) ) ;
#36124=CARTESIAN_POINT ( 'NONE',  ( -1.869488593554387679, -288.0507938011772353, -205.7095203647421329 ) ) ;
#36125=CARTESIAN_POINT ( 'NONE',  ( -34.29372919938526820, -281.8511042219344063, -196.3978499006769312 ) ) ;
#36126=CARTESIAN_POINT ( 'NONE',  ( 2.885484765620438985, -289.9491557817245848, -335.3876467558663990 ) ) ;
#36127=CARTESIAN_POINT ( 'NONE',  ( -12.36877165450719041, -290.0492890485820112, -342.7329635065437401 ) ) ;
#36128=CARTESIAN_POINT ( 'NONE',  ( -62.17351888655193193, -285.3750885767565819, -341.1857236781678466 ) ) ;
#36129=CARTESIAN_POINT ( 'NONE',  ( -112.7179820969497825, -278.9163410485656414, -254.5680578233979645 ) ) ;
#36131=CARTESIAN_POINT ( 'NONE',  ( 22.02481473602728457, -292.2692665478901972, -317.1251156490727681 ) ) ;
#36132=CARTESIAN_POINT ( 'NONE',  ( 37.33177405566786433, -281.1504378322624120, -251.5762235762069565 ) ) ;
#36133=CARTESIAN_POINT ( 'NONE',  ( -21.69642338203885146, -276.1152528934460975, -197.7932821805744936 ) ) ;
#36135=CARTESIAN_POINT ( 'NONE',  ( -85.33152481854864391, -287.9090924074130839, -210.2361428286349110 ) ) ;
#36136=CARTESIAN_POINT ( 'NONE',  ( 8.911505652960718393, -272.9167885492464620, -210.0733500168014700 ) ) ;
#36138=CARTESIAN_POINT ( 'NONE',  ( -11.71569465512919628, -279.9025552876253187, -201.8876143152286318 ) ) ;
#36139=CARTESIAN_POINT ( 'NONE',  ( 33.34120471936005714, -276.3781914395808599, -240.6956267869684893 ) ) ;
#36140=CARTESIAN_POINT ( 'NONE',  ( -55.45612375885657741, -299.2398894230291262, -198.9834729463937322 ) ) ;
#36141=CARTESIAN_POINT ( 'NONE',  ( -34.49971972426728684, -282.0759994322939406, -347.0731989144782688 ) ) ;
#36142=CARTESIAN_POINT ( 'NONE',  ( -99.15806731602999946, -292.8701305757792852, -229.5652703128246515 ) ) ;
#36143=CARTESIAN_POINT ( 'NONE',  ( -100.5564026171813765, -274.7197541196087514, -227.7190330620076111 ) ) ;
#36144=CARTESIAN_POINT ( 'NONE',  ( -104.9106396670619574, -298.2272803921481454, -234.1591187536167809 ) ) ;
#36145=CARTESIAN_POINT ( 'NONE',  ( -23.14671990896060549, -296.8704908393681308, -343.8887171170696320 ) ) ;
#36146=CARTESIAN_POINT ( 'NONE',  ( -62.16633697422399507, -281.3754123317987705, -341.0114909284214377 ) ) ;
#36147=CARTESIAN_POINT ( 'NONE',  ( -100.0113666966936421, -290.8111178333703606, -225.6592479574994172 ) ) ;
#36148=CARTESIAN_POINT ( 'NONE',  ( -5.811794039078424845, -272.4888846436464860, -202.7023282460580447 ) ) ;
#36149=CARTESIAN_POINT ( 'NONE',  ( 26.45670808654967843, -288.5990953131250194, -228.6933423732967299 ) ) ;
#36150=CARTESIAN_POINT ( 'NONE',  ( -102.6788527408748024, -289.9234544646740801, -237.0029979799479065 ) ) ;
#36152=CARTESIAN_POINT ( 'NONE',  ( -84.81292382985320444, -288.2664684170431428, -330.3042528901302148 ) ) ;
#36153=CARTESIAN_POINT ( 'NONE',  ( -45.36898666447230255, -288.8233762748753293, -342.9396971751189653 ) ) ;
#36155=CARTESIAN_POINT ( 'NONE',  ( -85.33023056062818057, -286.4861905406572760, -210.5397718275824275 ) ) ;
#36156=CARTESIAN_POINT ( 'NONE',  ( -80.82857180994611213, -277.9943416018773519, -329.0209805634548843 ) ) ;
#36157=CARTESIAN_POINT ( 'NONE',  ( 37.47930206118654439, -292.6845838309280907, -287.2521649463952826 ) ) ;
#36158=CARTESIAN_POINT ( 'NONE',  ( -79.09740938484608819, -284.2510563865067752, -334.9349016014886047 ) ) ;
#36159=CARTESIAN_POINT ( 'NONE',  ( -2.898492634936535861, -282.9427750701872810, -339.2191386595620202 ) ) ;
#36161=CARTESIAN_POINT ( 'NONE',  ( 2.712037078011438229, -280.9387457910447097, -209.2448531990257266 ) ) ;
#36162=CARTESIAN_POINT ( 'NONE',  ( 203.9604463576624198, 295.7236918480278405, -68.68622640684732517 ) ) ;
#36163=CARTESIAN_POINT ( 'NONE',  ( -114.3576317657223171, -272.4623070776191867, -284.0502682576448592 ) ) ;
#36164=CARTESIAN_POINT ( 'NONE',  ( 120.1367009602576843, 148.5113953528500588, -260.6353423530172790 ) ) ;
#36165=CARTESIAN_POINT ( 'NONE',  ( -99.41208178824524566, -272.2826807188951648, -231.6329699845104813 ) ) ;
#36166=CARTESIAN_POINT ( 'NONE',  ( 7.530922440670147822, -273.6013850210127885, -212.3897990701607057 ) ) ;
#36167=CARTESIAN_POINT ( 'NONE',  ( 1.732776325546617091, -294.0517974865024939, -336.6386571122970963 ) ) ;
#36168=CARTESIAN_POINT ( 'NONE',  ( 199.8274843008227322, 285.7222973586868306, -96.42357284835115649 ) ) ;
#36170=CARTESIAN_POINT ( 'NONE',  ( -94.70555265768811637, -271.9268954147405566, -219.7381321319227254 ) ) ;
#36171=CARTESIAN_POINT ( 'NONE',  ( -58.27540603824840559, -299.6391313150692781, -199.1386114633301361 ) ) ;
#36173=CARTESIAN_POINT ( 'NONE',  ( 36.04398846671895029, -288.8041319961679392, -265.5377609561448367 ) ) ;
#36175=CARTESIAN_POINT ( 'NONE',  ( -86.23620346047437124, -296.6529416620409734, -329.5400648823112419 ) ) ;
#36176=CARTESIAN_POINT ( 'NONE',  ( -71.21231322094249094, -286.0846060671940450, -205.6249610798599292 ) ) ;
#36177=CARTESIAN_POINT ( 'NONE',  ( -110.7372606567545148, -271.7548341422327667, -247.9404482524247726 ) ) ;
#36178=CARTESIAN_POINT ( 'NONE',  ( 25.58829341018716974, -294.9394667676555741, -314.4746136519703441 ) ) ;
#36179=CARTESIAN_POINT ( 'NONE',  ( -94.60158123103721550, -296.3464978079836101, -321.7697798333427386 ) ) ;
#36180=CARTESIAN_POINT ( 'NONE',  ( -110.3678558490410921, -290.7438610845713356, -268.4638771025769870 ) ) ;
#36182=CARTESIAN_POINT ( 'NONE',  ( -93.09948816549784567, -275.1792242776418220, -219.3480538221003542 ) ) ;
#36183=CARTESIAN_POINT ( 'NONE',  ( 31.49171079292095143, -274.7823020051932872, -304.0969182757463045 ) ) ;
#36185=CARTESIAN_POINT ( 'NONE',  ( -107.5225470536054218, -277.6553342928883126, -302.0213302858275028 ) ) ;
#36186=CARTESIAN_POINT ( 'NONE',  ( 17.89776309050611758, -273.2596508508046895, -221.3462019362630713 ) ) ;
#36187=CARTESIAN_POINT ( 'NONE',  ( -91.35957232452396681, -274.3402643619718333, -220.7815026719439118 ) ) ;
#36188=CARTESIAN_POINT ( 'NONE',  ( 0.7245659950945282368, -275.5146720957750404, -207.7962090360141758 ) ) ;
#36189=CARTESIAN_POINT ( 'NONE',  ( -5.558798911149763100, -276.2246234912205409, -201.3406774805418138 ) ) ;
#36190=CARTESIAN_POINT ( 'NONE',  ( 33.64288830939032238, -273.9001936931389878, -295.8049895631006621 ) ) ;
#36191=CARTESIAN_POINT ( 'NONE',  ( -101.5529013551746402, -296.7273134833705512, -305.3012711713106455 ) ) ;
#36192=CARTESIAN_POINT ( 'NONE',  ( 35.41778759416050804, -292.2754084186418027, -281.7116495838174046 ) ) ;
#36194=CARTESIAN_POINT ( 'NONE',  ( -114.3232277504436922, -279.0288211952927213, -271.6136572608987763 ) ) ;
#36195=CARTESIAN_POINT ( 'NONE',  ( -56.59812814241952594, -277.4739243381552569, -340.8280314783614813 ) ) ;
#36196=CARTESIAN_POINT ( 'NONE',  ( -21.07240359344990210, -284.9415278765324047, -195.6041232483434271 ) ) ;
#36197=CARTESIAN_POINT ( 'NONE',  ( -107.1945446413967602, -298.9146376392331490, -242.4612867527767435 ) ) ;
#36199=CARTESIAN_POINT ( 'NONE',  ( 33.54756173344362935, -286.5104435205909681, -252.2186946920048740 ) ) ;
#36200=CARTESIAN_POINT ( 'NONE',  ( -67.23217062761143836, -275.6894162747487371, -338.0703033919854192 ) ) ;
#36201=CARTESIAN_POINT ( 'NONE',  ( -71.94719444666444019, -276.0937830790541057, -335.3201917227514173 ) ) ;
#36202=CARTESIAN_POINT ( 'NONE',  ( -85.08664083924865906, -285.7108983820560297, -328.2672327651857245 ) ) ;
#36203=CARTESIAN_POINT ( 'NONE',  ( 20.34401482185246479, -277.3941091419751501, -315.7629543829226009 ) ) ;
#36206=CARTESIAN_POINT ( 'NONE',  ( 37.94210523876643038, -274.1050885672996174, -282.4726022670672592 ) ) ;
#36207=CARTESIAN_POINT ( 'NONE',  ( 19.93019163537890748, -275.5629893314053334, -224.9117720082027745 ) ) ;
#36208=CARTESIAN_POINT ( 'NONE',  ( -85.64652553884448594, -281.3861835362627062, -212.7026992079060221 ) ) ;
#36210=CARTESIAN_POINT ( 'NONE',  ( 36.11047487907135434, -289.6988326202091457, -288.1384983865893332 ) ) ;
#36211=CARTESIAN_POINT ( 'NONE',  ( 8.979508819043772405, -290.6871085107884483, -211.3098595550771961 ) ) ;
#36213=CARTESIAN_POINT ( 'NONE',  ( -40.51988780746840746, -296.8062553152834084, -197.0202687202381355 ) ) ;
#36214=CARTESIAN_POINT ( 'NONE',  ( -107.7351817500601499, -288.9995936178340230, -246.7894565015827482 ) ) ;
#36215=CARTESIAN_POINT ( 'NONE',  ( 126.6218730542261568, 145.9178657400643431, -262.1768218896158373 ) ) ;
#36217=CARTESIAN_POINT ( 'NONE',  ( -45.96680493742259443, -287.6393777948164256, -346.2314120663837684 ) ) ;
#36218=CARTESIAN_POINT ( 'NONE',  ( -36.55313339357986990, -284.3017864267904997, -194.3656720424375521 ) ) ;
#36219=CARTESIAN_POINT ( 'NONE',  ( -92.09138181866777018, -285.2790877378170649, -319.5516840566954215 ) ) ;
#36220=CARTESIAN_POINT ( 'NONE',  ( -108.8248672537759916, -285.5608388698738054, -254.7218818756450958 ) ) ;
#36221=CARTESIAN_POINT ( 'NONE',  ( -67.68998171193675262, -293.6358269726344474, -201.3732299545440299 ) ) ;
#36223=CARTESIAN_POINT ( 'NONE',  ( -15.78734953429887788, -274.6567307449877831, -196.4061723616887036 ) ) ;
#36224=CARTESIAN_POINT ( 'NONE',  ( -102.5679607563286453, -288.1249453047005886, -308.6071487640248847 ) ) ;
#36225=CARTESIAN_POINT ( 'NONE',  ( -75.33619964256796209, -277.5442842848946157, -337.3343813541747522 ) ) ;
#36227=CARTESIAN_POINT ( 'NONE',  ( 21.84241173838362471, -296.1582889395841676, -315.8692799580741735 ) ) ;
#36229=CARTESIAN_POINT ( 'NONE',  ( 31.95455697924148097, -295.6233781216988632, -236.9535640164627637 ) ) ;
#36230=CARTESIAN_POINT ( 'NONE',  ( -102.2143595042586384, -282.7682134834214480, -305.0061453710436581 ) ) ;
#36231=CARTESIAN_POINT ( 'NONE',  ( -58.70737429970168364, -277.7756543135695324, -198.4687775456655743 ) ) ;
#36232=CARTESIAN_POINT ( 'NONE',  ( -111.1426760980806421, -271.2793402925843225, -250.7651741823665930 ) ) ;
#36233=CARTESIAN_POINT ( 'NONE',  ( 29.24370265665852031, -275.3068144968546562, -300.5319118705396022 ) ) ;
#36234=CARTESIAN_POINT ( 'NONE',  ( 4.885234301560047676, -294.1539758710568435, -209.9032628039611836 ) ) ;
#36235=CARTESIAN_POINT ( 'NONE',  ( 34.71252335331385552, -294.3202420795350349, -257.1919305607589763 ) ) ;
#36236=CARTESIAN_POINT ( 'NONE',  ( 39.12197166903187906, -294.9765553017186903, -270.2922338149988377 ) ) ;
#36237=CARTESIAN_POINT ( 'NONE',  ( 29.15439281089968304, -295.3630349436596134, -308.3042450659706333 ) ) ;
#36238=CARTESIAN_POINT ( 'NONE',  ( -73.30425303103517365, -295.3767318592470588, -333.8882365478965539 ) ) ;
#36239=CARTESIAN_POINT ( 'NONE',  ( -109.6473059386526074, -292.2938767804967028, -290.4746084014727785 ) ) ;
#36240=CARTESIAN_POINT ( 'NONE',  ( -110.2239978041050108, -284.4058160186900750, -295.2040383013028304 ) ) ;
#36241=CARTESIAN_POINT ( 'NONE',  ( -67.02945677763784715, -271.8067254603124638, -200.6550021296810087 ) ) ;
#36242=CARTESIAN_POINT ( 'NONE',  ( 34.85496684569687176, -287.0470206597084939, -243.5909614202414559 ) ) ;
#36243=CARTESIAN_POINT ( 'NONE',  ( -109.4016682721986058, -280.2804856558169604, -289.8343764701360215 ) ) ;
#36244=CARTESIAN_POINT ( 'NONE',  ( 9.189192824204345911, -285.7684638311361596, -213.8077409972586338 ) ) ;
#36245=CARTESIAN_POINT ( 'NONE',  ( -62.12737906677441657, -287.3741381016166656, -341.2021366259628508 ) ) ;
#36246=CARTESIAN_POINT ( 'NONE',  ( -111.5035148913391652, -276.8895736657335078, -254.7960457309725371 ) ) ;
#36247=CARTESIAN_POINT ( 'NONE',  ( 64.33209501061345748, 48.33985520751024723, -319.1928417150128325 ) ) ;
#36248=CARTESIAN_POINT ( 'NONE',  ( -105.2734661674978582, -283.6987165151049908, -297.3924250609644560 ) ) ;
#36249=CARTESIAN_POINT ( 'NONE',  ( 1.161046873152622005, -281.7589742732415630, -204.0772676821704295 ) ) ;
#36250=CARTESIAN_POINT ( 'NONE',  ( -59.96938899550903557, -288.3971639252766295, -343.7151083917140681 ) ) ;
#36251=CARTESIAN_POINT ( 'NONE',  ( -108.8624574460518062, -280.4897720851660665, -243.9175747877524145 ) ) ;
#36252=CARTESIAN_POINT ( 'NONE',  ( -112.5775939159673413, -279.6916163650565181, -284.3203642132336313 ) ) ;
#36253=CARTESIAN_POINT ( 'NONE',  ( -69.73838228804767425, -279.4466036330701399, -204.9297293615757383 ) ) ;
#36254=CARTESIAN_POINT ( 'NONE',  ( 6.114281093487582197, -276.6245297572546633, -209.6060260265964530 ) ) ;
#36255=CARTESIAN_POINT ( 'NONE',  ( 37.08258354717888494, -293.3043273409497260, -250.5611721048423988 ) ) ;
#36256=CARTESIAN_POINT ( 'NONE',  ( 35.29596897621665619, -285.7940883196065442, -287.5546002946338717 ) ) ;
#36257=CARTESIAN_POINT ( 'NONE',  ( -92.24991617180027959, -292.8838006630689961, -217.4511133676278405 ) ) ;
#36258=CARTESIAN_POINT ( 'NONE',  ( -106.2825595604194007, -295.1400436662619313, -295.4380356678344697 ) ) ;
#36259=CARTESIAN_POINT ( 'NONE',  ( -0.5188315579235495134, -284.4788311169131134, -335.0557124160932290 ) ) ;
#36260=CARTESIAN_POINT ( 'NONE',  ( 18.84664950873154865, -293.8801406550237516, -316.9975506500848610 ) ) ;
#36261=CARTESIAN_POINT ( 'NONE',  ( -72.04473842588902244, -292.6838126011361396, -201.9565796498543193 ) ) ;
#36262=CARTESIAN_POINT ( 'NONE',  ( 32.07077971309043107, -281.8976896403491423, -247.2712957346687688 ) ) ;
#36263=EDGE_CURVE ( 'NONE', #51665, #85436, #67053, .T. ) ;
#36264=CARTESIAN_POINT ( 'NONE',  ( -106.6256940145609349, -272.0359502076033777, -237.3073980192059764 ) ) ;
#36265=CARTESIAN_POINT ( 'NONE',  ( -103.7062565986324074, -290.6960984426877417, -309.3130227035121607 ) ) ;
#36266=CARTESIAN_POINT ( 'NONE',  ( -107.0992998114111430, -282.3077402035950172, -300.0620126838579154 ) ) ;
#36267=CARTESIAN_POINT ( 'NONE',  ( -98.14029470744488037, -290.2547026373045469, -317.5763188062454674 ) ) ;
#36268=CARTESIAN_POINT ( 'NONE',  ( -8.250422995209902410, -286.7772066954727848, -203.3851142079568319 ) ) ;
#36270=CARTESIAN_POINT ( 'NONE',  ( 4.125645570873484047, -58.01712834443207356, -352.5247458089312431 ) ) ;
#36271=CARTESIAN_POINT ( 'NONE',  ( -12.70371226548575372, -92.33704762566186730, -356.1934519075916796 ) ) ;
#36272=CARTESIAN_POINT ( 'NONE',  ( -59.77344130751080797, -278.9512946298843303, -200.6699299088105306 ) ) ;
#36273=CARTESIAN_POINT ( 'NONE',  ( -41.05314201354045878, -278.9246709703813281, -197.1460152149548435 ) ) ;
#36274=CARTESIAN_POINT ( 'NONE',  ( 32.53565102784897078, -274.8041662142536552, -237.9402023170395921 ) ) ;
#36275=CARTESIAN_POINT ( 'NONE',  ( -75.47108427777141060, -209.2092562841938559, -354.8108879202522985 ) ) ;
#36277=CARTESIAN_POINT ( 'NONE',  ( -73.47089559995228569, -278.1572115865279216, -203.0165905177013883 ) ) ;
#36278=CARTESIAN_POINT ( 'NONE',  ( -96.43365694755391360, -281.9441096443633228, -315.9888705991562574 ) ) ;
#36279=CARTESIAN_POINT ( 'NONE',  ( -83.55097043383059940, -297.4358457569019833, -330.7488938313445601 ) ) ;
#36280=CARTESIAN_POINT ( 'NONE',  ( -83.87304728066754933, -291.8850398026606285, -214.0333080337985621 ) ) ;
#36281=CARTESIAN_POINT ( 'NONE',  ( -74.98277038719879783, -288.2496345354257983, -333.4979566671272551 ) ) ;
#36282=CARTESIAN_POINT ( 'NONE',  ( -58.10208276912891279, -274.4422983883305278, -196.2630790804410594 ) ) ;
#36283=CARTESIAN_POINT ( 'NONE',  ( -109.0460719088370922, -296.9003372973874662, -256.6020868879635941 ) ) ;
#36287=CARTESIAN_POINT ( 'NONE',  ( -112.2920192408740263, -280.5994772802668535, -260.3827359774746810 ) ) ;
#36288=CARTESIAN_POINT ( 'NONE',  ( 28.05093371741104846, -282.1824570015787117, -237.1120719176228135 ) ) ;
#36289=CARTESIAN_POINT ( 'NONE',  ( -6.660348339466530376, -282.2095739967647319, -200.8299252269443400 ) ) ;
#36291=CARTESIAN_POINT ( 'NONE',  ( 19.52718689039347666, -281.2619335770755242, -316.5256332902911254 ) ) ;
#36292=CARTESIAN_POINT ( 'NONE',  ( -82.05036154857259589, -281.2961159945497798, -211.0344171992517204 ) ) ;
#36293=CARTESIAN_POINT ( 'NONE',  ( -2.569570151768911792, -273.0007637543885721, -205.3872252979172117 ) ) ;
#36296=CARTESIAN_POINT ( 'NONE',  ( 23.39670155592854073, -276.9849378309200461, -317.4463042332989176 ) ) ;
#36298=CARTESIAN_POINT ( 'NONE',  ( 32.33589937920237389, -277.9153491264229388, -298.2507209485288513 ) ) ;
#36299=CARTESIAN_POINT ( 'NONE',  ( -14.78112057482514352, -275.3402855213526550, -343.4208032984566330 ) ) ;
#36302=CARTESIAN_POINT ( 'NONE',  ( -58.01086106323934644, -285.2976270958839677, -342.8805384401403558 ) ) ;
#36303=CARTESIAN_POINT ( 'NONE',  ( 14.99816214458775754, -292.0106829026373134, -219.1696597901038501 ) ) ;
#36304=CARTESIAN_POINT ( 'NONE',  ( 37.92544965862923334, -286.7026646452790715, -254.5439495920884951 ) ) ;
#36305=CARTESIAN_POINT ( 'NONE',  ( -108.7445966686949390, -282.5375701906197605, -289.8923581134595793 ) ) ;
#36306=CARTESIAN_POINT ( 'NONE',  ( -36.20246861896865909, -281.6123175184255274, -343.9415302566496280 ) ) ;
#36307=CARTESIAN_POINT ( 'NONE',  ( -5.154285822760023450, -284.5589061960181425, -203.2256437759452012 ) ) ;
#36308=CARTESIAN_POINT ( 'NONE',  ( 3.624500841363582637, -283.6928452341866773, -331.3233504130445226 ) ) ;
#36309=CARTESIAN_POINT ( 'NONE',  ( 32.85893579925581776, -273.2091214645902255, -243.9627967802626358 ) ) ;
#36310=CARTESIAN_POINT ( 'NONE',  ( -104.7151389405291013, -283.4177850857029171, -234.6495996259006347 ) ) ;
#36311=CARTESIAN_POINT ( 'NONE',  ( -33.51083836963886853, -297.0041143780780999, -345.2760001670768020 ) ) ;
#36312=CARTESIAN_POINT ( 'NONE',  ( -103.7989916403977446, -283.0178173581813894, -235.1291395622011464 ) ) ;
#36313=CARTESIAN_POINT ( 'NONE',  ( -102.3703112844064123, -279.9513551358339782, -236.5655819975815461 ) ) ;
#36315=CARTESIAN_POINT ( 'NONE',  ( 35.59164309125711867, -289.3192266991597990, -252.1744229241828634 ) ) ;
#36319=CARTESIAN_POINT ( 'NONE',  ( 38.21512075694161581, -295.4354221114915049, -267.4669025318149806 ) ) ;
#36320=CARTESIAN_POINT ( 'NONE',  ( -57.15233001207183605, -275.3074325462387719, -342.7513550718061310 ) ) ;
#36321=CARTESIAN_POINT ( 'NONE',  ( -97.17080362110569070, -289.1014366118644716, -318.5963624766644102 ) ) ;
#36322=CARTESIAN_POINT ( 'NONE',  ( -7.685326729214589037, -293.0567239932221923, -337.9539803973815424 ) ) ;
#36323=CARTESIAN_POINT ( 'NONE',  ( -110.8438349787734438, -277.2695470187993010, -267.8749848083858183 ) ) ;
#36324=CARTESIAN_POINT ( 'NONE',  ( -80.42599838442818339, -295.6008569065406277, -209.9077580954645157 ) ) ;
#36325=CARTESIAN_POINT ( 'NONE',  ( -69.24673890687128619, -292.9386211861154834, -204.1406347487781545 ) ) ;
#36326=CARTESIAN_POINT ( 'NONE',  ( -95.95921662488163406, -280.4090924074130839, -317.1477375740089997 ) ) ;
#36327=CARTESIAN_POINT ( 'NONE',  ( -67.96585304046065801, -293.9268371757372051, -340.2529559365293608 ) ) ;
#36328=CARTESIAN_POINT ( 'NONE',  ( -96.39636366464982586, -291.5374628736277032, -314.6426468297410679 ) ) ;
#36329=CARTESIAN_POINT ( 'NONE',  ( -97.53165900483173800, -289.4194283210287040, -223.9596579359920270 ) ) ;
#36330=CARTESIAN_POINT ( 'NONE',  ( -23.65794943948747431, -290.2992700861602771, -342.7190446257720282 ) ) ;
#36332=CARTESIAN_POINT ( 'NONE',  ( -90.70354437180714058, -290.6356243643067501, -320.4862157060960044 ) ) ;
#36333=FACE_OUTER_BOUND ( 'NONE', #40669, .T. ) ;
#36334=CARTESIAN_POINT ( 'NONE',  ( 7.713428883546115777, -289.6576352789380167, -332.3784887220405722 ) ) ;
#36335=CARTESIAN_POINT ( 'NONE',  ( -45.07886518987283608, -277.9748772883688730, -195.3523184816838238 ) ) ;
#36336=CARTESIAN_POINT ( 'NONE',  ( -112.0664190169488137, -279.1174459378747770, -251.8148457990174052 ) ) ;
#36337=CARTESIAN_POINT ( 'NONE',  ( 39.61968665131914236, -281.1776067918901276, -267.0625175803532443 ) ) ;
#36338=CARTESIAN_POINT ( 'NONE',  ( 17.45259208004352303, -284.8347823806874430, -219.1309666521230213 ) ) ;
#36340=CARTESIAN_POINT ( 'NONE',  ( 34.65931849064713077, -279.4565546235372153, -252.2340400334468598 ) ) ;
#36341=CARTESIAN_POINT ( 'NONE',  ( -46.24221349494202116, -283.9390585771792530, -195.8911138921568238 ) ) ;
#36343=CARTESIAN_POINT ( 'NONE',  ( -112.5498342827859375, -277.1948496265815152, -257.4597881898287710 ) ) ;
#36345=CARTESIAN_POINT ( 'NONE',  ( -106.3947958612632050, -283.9022967309953742, -236.9970283271693177 ) ) ;
#36346=CARTESIAN_POINT ( 'NONE',  ( -50.00635066727710409, -298.8278255376194465, -198.2291897246198289 ) ) ;
#36347=CARTESIAN_POINT ( 'NONE',  ( -107.7711184354598544, -292.4418267014910953, -248.2699836233372537 ) ) ;
#36348=CARTESIAN_POINT ( 'NONE',  ( -73.68076834684288201, -275.0051361215985253, -203.0856402590743244 ) ) ;
#36349=CARTESIAN_POINT ( 'NONE',  ( 34.64721688629088447, -275.0565429930813934, -258.0523117833445212 ) ) ;
#36350=CARTESIAN_POINT ( 'NONE',  ( -42.50260136110413356, -297.1174249626574806, -345.1833456158858553 ) ) ;
#36351=CARTESIAN_POINT ( 'NONE',  ( -99.86902646110527826, -290.1229547493315408, -315.3207015565205324 ) ) ;
#36352=CARTESIAN_POINT ( 'NONE',  ( 21.38827459945243348, -280.2818767912389717, -317.9220772282041594 ) ) ;
#36353=CARTESIAN_POINT ( 'NONE',  ( -11.15125625941679566, -292.2174285290663533, -197.8960977580323117 ) ) ;
#36355=CARTESIAN_POINT ( 'NONE',  ( -66.64725845036390695, -290.7173074597851610, -203.2448554221591621 ) ) ;
#36357=CARTESIAN_POINT ( 'NONE',  ( -0.4656461207899255106, -292.5618946539481726, -335.6840724772069393 ) ) ;
#36360=CARTESIAN_POINT ( 'NONE',  ( -107.0584599558214478, -290.3496887501069637, -248.4657962912532980 ) ) ;
#36362=CARTESIAN_POINT ( 'NONE',  ( 9.657213943495289499, -287.6224896700454678, -209.6657945352397121 ) ) ;
#36363=CARTESIAN_POINT ( 'NONE',  ( -37.37352853689063181, -300.5519495502701375, -200.3611179825600459 ) ) ;
#36364=CARTESIAN_POINT ( 'NONE',  ( -69.44048843942523774, -294.5230718174798312, -340.1070506103724256 ) ) ;
#36365=CARTESIAN_POINT ( 'NONE',  ( -113.8611157496324751, -285.8359972113440222, -272.8500083645006384 ) ) ;
#36366=CARTESIAN_POINT ( 'NONE',  ( -108.9799035729099614, -284.2003328795066750, -284.3956401234800069 ) ) ;
#36367=CARTESIAN_POINT ( 'NONE',  ( -13.54335403933255400, -278.2577663074001748, -340.1596332506368867 ) ) ;
#36368=CARTESIAN_POINT ( 'NONE',  ( 27.20253989103627745, -292.0753591847402504, -307.8562894171354856 ) ) ;
#36369=CARTESIAN_POINT ( 'NONE',  ( 20.49953952209563823, -295.9558177055138799, -316.5588679779123709 ) ) ;
#36370=CARTESIAN_POINT ( 'NONE',  ( 12.00336940515391859, -275.1430749594844656, -324.7641723426035583 ) ) ;
#36373=CARTESIAN_POINT ( 'NONE',  ( -19.29635662870749968, -294.4929693733215004, -345.2498696573192092 ) ) ;
#36374=CARTESIAN_POINT ( 'NONE',  ( 32.76361034346400913, -289.7991338785600988, -295.3922913539431647 ) ) ;
#36375=CARTESIAN_POINT ( 'NONE',  ( -54.90415217815425564, -295.8263339674465442, -197.3935939614778761 ) ) ;
#36376=CARTESIAN_POINT ( 'NONE',  ( -3.593475819944103922, -299.5450462478421514, -193.6641989976668299 ) ) ;
#36377=CARTESIAN_POINT ( 'NONE',  ( 27.74512343043636164, -287.7506908613603969, -236.9689384534894430 ) ) ;
#36379=CARTESIAN_POINT ( 'NONE',  ( -59.60824655745756928, -276.3924387684125463, -343.8255387760003714 ) ) ;
#36380=CARTESIAN_POINT ( 'NONE',  ( -79.41425143792584151, -296.2557669218658134, -334.7289143769236830 ) ) ;
#36381=CARTESIAN_POINT ( 'NONE',  ( -6.156899895186679572, -286.7863184127784280, -339.4104750969341922 ) ) ;
#36382=CARTESIAN_POINT ( 'NONE',  ( -36.27048488967021456, -295.3723825001221144, -347.3456204804983827 ) ) ;
#36383=CARTESIAN_POINT ( 'NONE',  ( -66.57643662309044430, -291.9916345885015403, -203.4476091154623703 ) ) ;
#36387=CARTESIAN_POINT ( 'NONE',  ( -37.99609804505431043, -287.5642081643197230, -194.0572549159202538 ) ) ;
#36388=CARTESIAN_POINT ( 'NONE',  ( 25.18497378105905682, -285.6952119285918457, -320.2651865833026363 ) ) ;
#36390=CARTESIAN_POINT ( 'NONE',  ( -97.61182796767998582, -278.5406794153579426, -222.6031398282109990 ) ) ;
#36391=CARTESIAN_POINT ( 'NONE',  ( -48.57947521258299162, -285.1957341605266834, -344.3458517822152771 ) ) ;
#36392=CARTESIAN_POINT ( 'NONE',  ( -112.5602352529624568, -282.9537688751075279, -284.0973899021352054 ) ) ;
#36393=CARTESIAN_POINT ( 'NONE',  ( 23.11723423016862000, -286.2273906548497280, -313.7895816412628847 ) ) ;
#36394=CARTESIAN_POINT ( 'NONE',  ( 35.31577387817176117, -277.6868993481881489, -291.8824373098256046 ) ) ;
#36395=CARTESIAN_POINT ( 'NONE',  ( -91.89501436541394241, -297.7388628330472784, -221.7614847793745412 ) ) ;
#36397=CARTESIAN_POINT ( 'NONE',  ( -42.44054460876731127, -293.8026256444777573, -343.6771821389189654 ) ) ;
#36398=CARTESIAN_POINT ( 'NONE',  ( -64.71381235846634183, -280.3554992246197344, -198.4434247771710886 ) ) ;
#36399=CARTESIAN_POINT ( 'NONE',  ( -109.6218116890025271, -278.6916863063167966, -259.7836677673691383 ) ) ;
#36400=CARTESIAN_POINT ( 'NONE',  ( -91.36656658136038800, -278.6059421941404253, -221.1147326024030519 ) ) ;
#36401=CARTESIAN_POINT ( 'NONE',  ( -60.78974241462493211, -274.8346646958725046, -197.2873410775770537 ) ) ;
#36402=CARTESIAN_POINT ( 'NONE',  ( -38.55391650943938942, -275.9873527451235873, -347.0424262818040120 ) ) ;
#36403=CARTESIAN_POINT ( 'NONE',  ( -84.59855605908614962, -218.1032794253833345, -349.8295654733143465 ) ) ;
#36405=CARTESIAN_POINT ( 'NONE',  ( -90.29058621344924518, -297.2085371877467992, -325.5249781917722771 ) ) ;
#36407=DIRECTION ( 'NONE',  ( -0.000000000000000000, 1.000000000000000000, 1.224646799147353207E-16 ) ) ;
#36408=CARTESIAN_POINT ( 'NONE',  ( -101.2675758579773628, -286.1219871243400803, -234.3723955102004481 ) ) ;
#36409=CARTESIAN_POINT ( 'NONE',  ( -62.88221399330386419, -287.4842605982757391, -198.7953708380715625 ) ) ;
#36410=CARTESIAN_POINT ( 'NONE',  ( 10.17523427537661895, -287.7253086583515369, -325.9801229707090329 ) ) ;
#36411=CARTESIAN_POINT ( 'NONE',  ( -4.196030428723147132, -282.1344808644357158, -339.8082347460974688 ) ) ;
#36412=CARTESIAN_POINT ( 'NONE',  ( -107.9870926799286082, -277.2315822329670141, -249.0147148451659973 ) ) ;
#36413=CARTESIAN_POINT ( 'NONE',  ( -110.1870792805642623, -286.2271010746590036, -284.6585379884362510 ) ) ;
#36414=CARTESIAN_POINT ( 'NONE',  ( -54.63690488973530535, -278.3058510332486435, -198.6733560630677573 ) ) ;
#36415=CARTESIAN_POINT ( 'NONE',  ( -45.94934448409083672, -278.4786179343786330, -343.3994261518290614 ) ) ;
#36416=CARTESIAN_POINT ( 'NONE',  ( 0.6391080398062483070, -275.0658396896797058, -207.9476046015776092 ) ) ;
#36417=CARTESIAN_POINT ( 'NONE',  ( 23.81588913860320744, -286.9645263509295887, -316.4887452234615921 ) ) ;
#36418=CARTESIAN_POINT ( 'NONE',  ( -71.65743201224400138, -284.2968648249295711, -339.1113133748129940 ) ) ;
#36419=CARTESIAN_POINT ( 'NONE',  ( 19.74206998457583495, -282.7462015964781585, -322.0236625296275292 ) ) ;
#36423=CARTESIAN_POINT ( 'NONE',  ( -9.986839191855487741, -290.5591411672682511, -341.0153256683562972 ) ) ;
#36424=CARTESIAN_POINT ( 'NONE',  ( -87.07664730730149927, -288.4124882830251408, -328.5661898010961295 ) ) ;
#36425=CARTESIAN_POINT ( 'NONE',  ( -37.13892041667711652, -297.2519284402460471, -197.1968135573092695 ) ) ;
#36426=CARTESIAN_POINT ( 'NONE',  ( 36.60842445409088697, -292.6355088390661194, -249.2254012382605026 ) ) ;
#36427=CARTESIAN_POINT ( 'NONE',  ( -20.99418713197473707, -287.3184175860797609, -342.2183832333910800 ) ) ;
#36428=CARTESIAN_POINT ( 'NONE',  ( 22.12749083094972136, -292.4013691240335788, -314.4223179443346226 ) ) ;
#36429=CARTESIAN_POINT ( 'NONE',  ( 33.76947212699940337, -288.5180270808524483, -252.1354027589475777 ) ) ;
#36430=CARTESIAN_POINT ( 'NONE',  ( 35.78497577281001440, -296.2662352645559167, -287.0191576251351080 ) ) ;
#36431=CARTESIAN_POINT ( 'NONE',  ( 34.05194201517003449, -289.8489573497968195, -293.3382481384838343 ) ) ;
#36432=CARTESIAN_POINT ( 'NONE',  ( -106.6662369310979130, -288.9305696963664900, -241.3070817583218002 ) ) ;
#36434=CARTESIAN_POINT ( 'NONE',  ( -112.3862957294052478, -292.5394277079515177, -271.3649819998132671 ) ) ;
#36435=CARTESIAN_POINT ( 'NONE',  ( -108.2595005624916951, -285.7339114465795546, -252.0834258337313258 ) ) ;
#36436=CARTESIAN_POINT ( 'NONE',  ( -6.659168104624491491, -294.4541666545368912, -201.7278554629307621 ) ) ;
#36439=CARTESIAN_POINT ( 'NONE',  ( -112.6969001285957006, -274.5317257255920822, -270.3862698198935846 ) ) ;
#36440=CARTESIAN_POINT ( 'NONE',  ( -3.555882753585494882, -281.7914482473875069, -335.2682982919924939 ) ) ;
#36441=CARTESIAN_POINT ( 'NONE',  ( -54.16233559640447481, -281.2678529830369030, -343.5040780991286056 ) ) ;
#36442=CARTESIAN_POINT ( 'NONE',  ( -44.79016990575826895, -294.3411911617103556, -346.8910703211512327 ) ) ;
#36443=CARTESIAN_POINT ( 'NONE',  ( 31.12057963426378748, -273.4186716975830791, -242.1036699288960961 ) ) ;
#36444=CARTESIAN_POINT ( 'NONE',  ( -81.69661911889993178, -275.7412690584095571, -330.1436853111102891 ) ) ;
#36445=CARTESIAN_POINT ( 'NONE',  ( -110.5892369044117061, -297.7808603486535048, -276.9604793670855543 ) ) ;
#36446=CARTESIAN_POINT ( 'NONE',  ( -38.33143454498044633, -272.6147074871836367, -193.9567547502762466 ) ) ;
#36447=CARTESIAN_POINT ( 'NONE',  ( 33.87388428204629776, -294.7346217578486858, -251.8215533801229640 ) ) ;
#36448=CARTESIAN_POINT ( 'NONE',  ( 82.64890176555634582, -299.5541904835127980, -193.4651424135224147 ) ) ;
#36449=CARTESIAN_POINT ( 'NONE',  ( -9.159250691535568478, -295.4768390451197888, -337.8903180535593833 ) ) ;
#36451=CARTESIAN_POINT ( 'NONE',  ( 36.12190479245951025, -285.3571910632523441, -253.5256369598023980 ) ) ;
#36452=CARTESIAN_POINT ( 'NONE',  ( -107.6028088719952649, -296.2903010737892373, -290.1696161102805718 ) ) ;
#36453=CARTESIAN_POINT ( 'NONE',  ( -108.2271400225182134, -284.1678567040683561, -300.5683431800719063 ) ) ;
#36454=CARTESIAN_POINT ( 'NONE',  ( 33.84149516489766540, -286.8448202923074746, -240.9183114128727539 ) ) ;
#36455=CARTESIAN_POINT ( 'NONE',  ( 35.43658105321669183, -291.3272050204694779, -252.8893424519120856 ) ) ;
#36456=CARTESIAN_POINT ( 'NONE',  ( -7.590052577300235193, -279.6295167762784786, -199.5019549692357828 ) ) ;
#36457=CARTESIAN_POINT ( 'NONE',  ( -69.91165696735023971, -274.9809262143061233, -337.9199732462171255 ) ) ;
#36459=CARTESIAN_POINT ( 'NONE',  ( 31.35162347390982163, -286.0022478705710114, -244.3649491040047224 ) ) ;
#36460=CARTESIAN_POINT ( 'NONE',  ( -62.67457298357670226, -288.2944788387416679, -342.8033148382984336 ) ) ;
#36463=CARTESIAN_POINT ( 'NONE',  ( -97.04372138491163469, -297.5514353866338411, -313.7659610498172356 ) ) ;
#36464=CARTESIAN_POINT ( 'NONE',  ( -38.18177614580379498, -281.4670832233994133, -193.9549626837489598 ) ) ;
#36465=CARTESIAN_POINT ( 'NONE',  ( -108.2935150985727830, -294.8996634671069046, -244.9791016358023796 ) ) ;
#36466=CARTESIAN_POINT ( 'NONE',  ( 34.58865079827489808, -281.0530422292969206, -257.7868544879223123 ) ) ;
#36467=CARTESIAN_POINT ( 'NONE',  ( 24.88753236352268061, -294.3209627146312641, -315.7322275433445498 ) ) ;
#36469=CARTESIAN_POINT ( 'NONE',  ( -108.6561274243400419, -280.8541387050315734, -246.9742846930662381 ) ) ;
#36470=CARTESIAN_POINT ( 'NONE',  ( -92.91515624540760143, -296.2879147817570811, -222.6448787601670745 ) ) ;
#36473=CARTESIAN_POINT ( 'NONE',  ( -69.69987050817832142, -285.4601682883286458, -337.6418301774566544 ) ) ;
#36475=CARTESIAN_POINT ( 'NONE',  ( -37.30987171927208834, -283.5523547857346784, -195.3611179825600175 ) ) ;
#36476=CARTESIAN_POINT ( 'NONE',  ( 26.80140507305364395, -274.1918399145835110, -228.0548433232394814 ) ) ;
#36477=CARTESIAN_POINT ( 'NONE',  ( -109.6998281673912459, -290.5178377968475161, -260.3270114090263974 ) ) ;
#36478=CARTESIAN_POINT ( 'NONE',  ( 35.39094872883214293, -283.2272651635992133, -282.2215371733696543 ) ) ;
#36479=CARTESIAN_POINT ( 'NONE',  ( -94.40985545298124748, -274.8081166465035494, -223.5474842818036052 ) ) ;
#36480=CARTESIAN_POINT ( 'NONE',  ( -52.73586600945811398, -284.8462156810082888, -345.0438560502974497 ) ) ;
#36481=CARTESIAN_POINT ( 'NONE',  ( 36.09993931412886781, -280.3598372342331686, -271.3342546248802023 ) ) ;
#36482=CARTESIAN_POINT ( 'NONE',  ( -93.72846963032985457, -281.2394580579449439, -220.8892438720545499 ) ) ;
#36483=CARTESIAN_POINT ( 'NONE',  ( -102.7201589957636543, -273.2509871067296672, -229.6836411608153412 ) ) ;
#36484=CARTESIAN_POINT ( 'NONE',  ( -21.35271907222038124, -274.0850939294836621, -195.0394578224199051 ) ) ;
#36485=CARTESIAN_POINT ( 'NONE',  ( 30.03161579577744789, -295.0515150704758867, -238.5827869729036195 ) ) ;
#36486=CARTESIAN_POINT ( 'NONE',  ( 129.9467878515196162, -299.5541904835127980, -195.3611179825600175 ) ) ;
#36489=CARTESIAN_POINT ( 'NONE',  ( -27.92522668614256531, -293.0735382079603824, -345.5909149364619566 ) ) ;
#36490=CARTESIAN_POINT ( 'NONE',  ( -63.32274966100137448, -273.2119769330540180, -202.0616450105656838 ) ) ;
#36492=CARTESIAN_POINT ( 'NONE',  ( -74.35964818113419028, -293.0891981603970180, -203.6349666226969362 ) ) ;
#36493=CARTESIAN_POINT ( 'NONE',  ( -95.99890600148557951, -275.6948066931273615, -223.6242672951989618 ) ) ;
#36494=CARTESIAN_POINT ( 'NONE',  ( 17.19607135086742744, -294.0138978930153257, -216.4938751055042587 ) ) ;
#36495=CARTESIAN_POINT ( 'NONE',  ( 27.29204555773020147, -290.0584838156564160, -308.1797603603603761 ) ) ;
#36496=CARTESIAN_POINT ( 'NONE',  ( -81.93169923006281863, -275.6612755205580925, -330.4590414379638332 ) ) ;
#36497=CARTESIAN_POINT ( 'NONE',  ( -96.40085331815474490, -279.8470819201439213, -315.6748093526999810 ) ) ;
#36498=CARTESIAN_POINT ( 'NONE',  ( -17.86686179102301963, -292.8789093712503018, -342.2084900074823963 ) ) ;
#36499=CARTESIAN_POINT ( 'NONE',  ( 24.92886264784288741, -283.9922253867258064, -313.5427504955195559 ) ) ;
#36501=CARTESIAN_POINT ( 'NONE',  ( -101.7918859083870728, -283.7499483021175024, -304.7945536219049245 ) ) ;
#36502=CARTESIAN_POINT ( 'NONE',  ( -71.11092043020893527, -280.6965132133107090, -201.5052375403541305 ) ) ;
#36503=CARTESIAN_POINT ( 'NONE',  ( -85.86277093032305174, -282.5022165188523786, -329.6377103750797346 ) ) ;
#36504=CARTESIAN_POINT ( 'NONE',  ( -68.58776078581355762, -280.5927399623715246, -200.2289890805708410 ) ) ;
#36507=CARTESIAN_POINT ( 'NONE',  ( 31.91557222956466333, -276.6572711153784780, -238.2019694202430173 ) ) ;
#36508=CARTESIAN_POINT ( 'NONE',  ( -92.08974858914540107, -293.6948066931273047, -226.7417163044926838 ) ) ;
#36510=CARTESIAN_POINT ( 'NONE',  ( -104.8701366780603053, -274.9777367177613314, -238.1130377222687287 ) ) ;
#36511=CARTESIAN_POINT ( 'NONE',  ( -100.5817118619040400, -276.0356198849154339, -310.1130789898172679 ) ) ;
#36512=CARTESIAN_POINT ( 'NONE',  ( -99.21907647818083831, -292.9042021024465043, -226.2571010356958539 ) ) ;
#36513=CARTESIAN_POINT ( 'NONE',  ( 34.16555331793885131, -293.1015729161529748, -285.6068254659196555 ) ) ;
#36514=CARTESIAN_POINT ( 'NONE',  ( -62.74925240929006520, -288.8817083902563922, -343.0396539042784525 ) ) ;
#36516=CARTESIAN_POINT ( 'NONE',  ( 38.85486018996409996, -292.0548243258436401, -264.6435584202449718 ) ) ;
#36517=CARTESIAN_POINT ( 'NONE',  ( -94.04973101028605242, -282.2891591118892052, -317.5907659872622730 ) ) ;
#36518=CARTESIAN_POINT ( 'NONE',  ( -70.50328470984743490, -291.3544868212671304, -336.7918843677855421 ) ) ;
#36519=CARTESIAN_POINT ( 'NONE',  ( 17.98709336804638426, -283.5528532863116880, -318.7343346335289880 ) ) ;
#36520=CARTESIAN_POINT ( 'NONE',  ( -54.43751496834735804, -290.2077171707551315, -345.2525055622558057 ) ) ;
#36521=CARTESIAN_POINT ( 'NONE',  ( 18.87944378451639338, -281.3831051958953822, -223.6815336760596722 ) ) ;
#36522=CARTESIAN_POINT ( 'NONE',  ( -19.39527459654731345, -293.6213151031814732, -344.8867495324243464 ) ) ;
#36523=CARTESIAN_POINT ( 'NONE',  ( 12.31926571097654133, -289.1836920822031516, -328.9951293747710110 ) ) ;
#36524=CARTESIAN_POINT ( 'NONE',  ( -20.50376113063230932, -289.3339898784125808, -345.4891115516581976 ) ) ;
#36525=CARTESIAN_POINT ( 'NONE',  ( -96.57606785617630862, -285.3157047089517846, -227.6749393446403644 ) ) ;
#36528=CARTESIAN_POINT ( 'NONE',  ( -32.07434690690416090, -296.8468130020423814, -345.9556422431013516 ) ) ;
#36529=CARTESIAN_POINT ( 'NONE',  ( -76.84206035037567517, -294.2538731055311132, -335.9438991138271149 ) ) ;
#36531=CARTESIAN_POINT ( 'NONE',  ( -93.26212900985719045, -278.2810089578179031, -223.0521492308486700 ) ) ;
#36532=CARTESIAN_POINT ( 'NONE',  ( -85.76463616281066038, -272.9096813799963002, -210.5719369476023246 ) ) ;
#36533=CARTESIAN_POINT ( 'NONE',  ( -90.92454900864993306, -294.3095183062736169, -321.0269811628870116 ) ) ;
#36534=CARTESIAN_POINT ( 'NONE',  ( 36.71310783501684227, -277.3281547737376513, -271.5795866355633734 ) ) ;
#36535=CARTESIAN_POINT ( 'NONE',  ( 53.24685640498476857, -297.4411105498125494, -196.3754083438691680 ) ) ;
#36536=CARTESIAN_POINT ( 'NONE',  ( 34.03030215777685896, -294.5319224616985707, -253.1853297622871253 ) ) ;
#36537=CARTESIAN_POINT ( 'NONE',  ( -107.8965870705577714, -297.3697980464898478, -290.2667453949376295 ) ) ;
#36539=CARTESIAN_POINT ( 'NONE',  ( -81.86368492034900157, -295.4474594603536275, -209.7339231300119309 ) ) ;
#36540=CARTESIAN_POINT ( 'NONE',  ( -43.29015940290972253, -298.6304444905814535, -193.6403276531499102 ) ) ;
#36541=CARTESIAN_POINT ( 'NONE',  ( -111.8761160808900712, -274.6594503038225525, -262.0171689033327311 ) ) ;
#36542=CARTESIAN_POINT ( 'NONE',  ( -50.78292581272314266, -290.1692093377737365, -342.4042244765716987 ) ) ;
#36543=CARTESIAN_POINT ( 'NONE',  ( -55.80455848221016879, -295.6296250512015718, -341.0620141482948497 ) ) ;
#36544=CARTESIAN_POINT ( 'NONE',  ( -106.0654729793480016, -280.1271758439433484, -301.3983442815521130 ) ) ;
#36545=CARTESIAN_POINT ( 'NONE',  ( -113.8917448642033463, -277.2215908492424887, -271.5836930016295696 ) ) ;
#36546=CARTESIAN_POINT ( 'NONE',  ( -1.688774056714934524, -281.9407952177457446, -338.4946754226625671 ) ) ;
#36547=CARTESIAN_POINT ( 'NONE',  ( 32.46401906989120079, -274.4860853738308037, -237.9779001241196568 ) ) ;
#36548=CARTESIAN_POINT ( 'NONE',  ( -64.60509204537189021, -281.4907336159563442, -339.6288713715461540 ) ) ;
#36549=CARTESIAN_POINT ( 'NONE',  ( -81.75587349860425945, -277.8582113541465333, -208.4432561216914621 ) ) ;
#36550=CARTESIAN_POINT ( 'NONE',  ( -85.60753638395715370, -277.3865062877884498, -212.6700588687814957 ) ) ;
#36551=CARTESIAN_POINT ( 'NONE',  ( -103.7288933501302637, -271.5528551873201764, -238.6102834815369533 ) ) ;
#36552=CARTESIAN_POINT ( 'NONE',  ( -1.924503310254754851, -278.5832811827476121, -336.4861826383494758 ) ) ;
#36555=CARTESIAN_POINT ( 'NONE',  ( 18.22031444830711067, -290.8646583116623106, -219.4566060044820688 ) ) ;
#36557=CARTESIAN_POINT ( 'NONE',  ( -51.68530585684888479, -289.2307918871019865, -346.0133550591836524 ) ) ;
#36558=CARTESIAN_POINT ( 'NONE',  ( -5.904785239958090237, -276.4646039017158046, -202.0841173688888830 ) ) ;
#36559=CARTESIAN_POINT ( 'NONE',  ( -91.62711212189105936, -271.2786216151463350, -218.5920247042811866 ) ) ;
#36560=CARTESIAN_POINT ( 'NONE',  ( -99.20813169897998307, -284.3570358326381324, -224.7027244813578761 ) ) ;
#36563=CARTESIAN_POINT ( 'NONE',  ( -85.12579157651852313, -281.7112199555536449, -328.2349310359689980 ) ) ;
#36565=CARTESIAN_POINT ( 'NONE',  ( 22.92268566804259677, -291.7660446965438155, -228.4422569640934455 ) ) ;
#36566=CARTESIAN_POINT ( 'NONE',  ( -22.18487566183325654, -284.3877777815829404, -197.6369298623386896 ) ) ;
#36569=CARTESIAN_POINT ( 'NONE',  ( 24.24440325228689019, -290.9710883034318272, -227.5348283827006526 ) ) ;
#36570=CARTESIAN_POINT ( 'NONE',  ( -67.62416511008005671, -281.9222153161818483, -340.4016781501875926 ) ) ;
#36571=CARTESIAN_POINT ( 'NONE',  ( -41.88570400320441678, -278.7104610007943961, -344.0338310570593876 ) ) ;
#36572=CARTESIAN_POINT ( 'NONE',  ( -105.4241671716930995, -285.3010193932071843, -305.5878671253857419 ) ) ;
#36573=CARTESIAN_POINT ( 'NONE',  ( -98.10706653902032315, -285.1137375108239098, -229.9065725649641365 ) ) ;
#36574=CARTESIAN_POINT ( 'NONE',  ( -51.37562253531062595, -278.6604086069558548, -342.5997775589087837 ) ) ;
#36575=CARTESIAN_POINT ( 'NONE',  ( -110.5130208671179020, -279.3872127908599623, -267.9130364060530383 ) ) ;
#36577=CARTESIAN_POINT ( 'NONE',  ( -79.82680273196537257, -287.4782616354280549, -208.4921339988828208 ) ) ;
#36579=CARTESIAN_POINT ( 'NONE',  ( -109.4382868577820886, -296.0417583861024582, -297.5500918960469221 ) ) ;
#36580=CARTESIAN_POINT ( 'NONE',  ( 33.89065833062556976, -289.8232291058309329, -292.8447225331511845 ) ) ;
#36582=CARTESIAN_POINT ( 'NONE',  ( 13.84574458161073096, -284.9090924074130839, -334.4957818155094174 ) ) ;
#36584=CARTESIAN_POINT ( 'NONE',  ( 32.67336439791520775, -292.3406053428197424, -300.5663890819524227 ) ) ;
#36585=CARTESIAN_POINT ( 'NONE',  ( 7.332005941075407485, -288.1935156473381880, -211.6880588197431052 ) ) ;
#36586=CARTESIAN_POINT ( 'NONE',  ( -108.2036977293781206, -280.5913093958762943, -248.9940566479791073 ) ) ;
#36587=CARTESIAN_POINT ( 'NONE',  ( 21.95943204025457263, -289.6290520084179434, -318.5686651770561753 ) ) ;
#36588=CARTESIAN_POINT ( 'NONE',  ( -69.85372365634481184, -285.4804333070601956, -337.9620477735047643 ) ) ;
#36589=CARTESIAN_POINT ( 'NONE',  ( -112.4839403549753740, -278.5085738127202717, -287.1731297069448487 ) ) ;
#36591=CARTESIAN_POINT ( 'NONE',  ( 28.31113909985324639, -292.1282277802108638, -307.8702154671547078 ) ) ;
#36592=CARTESIAN_POINT ( 'NONE',  ( 12.99377416014388054, -280.5661413056571405, -212.0915716254347956 ) ) ;
#36593=CARTESIAN_POINT ( 'NONE',  ( -62.46971173697773594, -275.5821315465273642, -200.5080685700372101 ) ) ;
#36595=CARTESIAN_POINT ( 'NONE',  ( -85.33152481854864391, -293.9090924074130839, -210.2361428286349110 ) ) ;
#36596=CARTESIAN_POINT ( 'NONE',  ( -94.31169722839038627, -271.4820000931889581, -220.0779851703954932 ) ) ;
#36598=CARTESIAN_POINT ( 'NONE',  ( -54.50116472288227243, -279.3334604347061827, -199.2909844019335424 ) ) ;
#36599=CARTESIAN_POINT ( 'NONE',  ( 37.52092034518254593, -276.9620950208469594, -286.6581229933371446 ) ) ;
#36600=CARTESIAN_POINT ( 'NONE',  ( -70.75114926502246249, -299.0278412241978003, -204.7789325566142509 ) ) ;
#36601=CARTESIAN_POINT ( 'NONE',  ( -37.32636916822458062, -282.1106815811281763, -347.1388483921566603 ) ) ;
#36602=CARTESIAN_POINT ( 'NONE',  ( -88.64898494609887791, -293.0808336801002270, -216.9466971967346183 ) ) ;
#36603=CARTESIAN_POINT ( 'NONE',  ( -72.97425534808641601, -299.1092219085675765, -202.8266578592474900 ) ) ;
#36604=CARTESIAN_POINT ( 'NONE',  ( -82.74762329647232662, -298.6521798275545621, -208.5998954309416149 ) ) ;
#36605=CARTESIAN_POINT ( 'NONE',  ( -20.40918813156419276, -296.8344807796837017, -343.3070488997238385 ) ) ;
#36606=CARTESIAN_POINT ( 'NONE',  ( -54.12501131020716372, -281.2678529809568886, -343.3415255826482166 ) ) ;
#36607=CARTESIAN_POINT ( 'NONE',  ( -104.6782312795411372, -270.9983245579026061, -238.1487232867053194 ) ) ;
#36608=CARTESIAN_POINT ( 'NONE',  ( -69.47425100821460831, -287.2364620996675058, -201.2531989504296348 ) ) ;
#36609=CARTESIAN_POINT ( 'NONE',  ( -23.74125767497766404, -287.7947294931971669, -342.4495110409590666 ) ) ;
#36610=CARTESIAN_POINT ( 'NONE',  ( -106.2395333457863842, -263.2123202082037210, -317.5511267182615711 ) ) ;
#36612=CARTESIAN_POINT ( 'NONE',  ( -98.72036414668833970, -289.7368448932155616, -224.8280436247866021 ) ) ;
#36613=CARTESIAN_POINT ( 'NONE',  ( 7.989752088668538477, -288.0793214224137273, -327.6074884054769996 ) ) ;
#36615=CARTESIAN_POINT ( 'NONE',  ( -107.6482779210042082, -286.0254304302478658, -239.5936985957671652 ) ) ;
#36616=CARTESIAN_POINT ( 'NONE',  ( -95.28720915859398133, -278.2604657757648283, -314.7954005812092078 ) ) ;
#36617=CARTESIAN_POINT ( 'NONE',  ( 19.19710981558070273, -291.7647337768821671, -218.5455268920495087 ) ) ;
#36618=CARTESIAN_POINT ( 'NONE',  ( -111.3910719121094104, -284.9433730509019256, -291.0976395125927638 ) ) ;
#36619=CARTESIAN_POINT ( 'NONE',  ( 38.49145981554141116, -282.9593322185109514, -261.4118835478699907 ) ) ;
#36620=CARTESIAN_POINT ( 'NONE',  ( -35.89533557317339074, -283.3677901277861793, -347.3394982626378464 ) ) ;
#36621=CARTESIAN_POINT ( 'NONE',  ( 31.99534397646523232, -281.5796089010634091, -247.3006495722195837 ) ) ;
#36622=CARTESIAN_POINT ( 'NONE',  ( 203.7386562182569207, 295.8239156117444395, -54.00000000004033041 ) ) ;
#36624=CARTESIAN_POINT ( 'NONE',  ( -29.49651792000635098, -278.9528598573265867, -344.8342786300242437 ) ) ;
#36625=CARTESIAN_POINT ( 'NONE',  ( -32.21414366731176671, -123.8110585969327246, -363.4835760948135430 ) ) ;
#36626=CARTESIAN_POINT ( 'NONE',  ( -94.98170178195216806, -238.2700655660910911, -338.7697016782443029 ) ) ;
#36627=CARTESIAN_POINT ( 'NONE',  ( -100.8528764064363088, -272.2470669890015529, -233.9421604980510949 ) ) ;
#36628=CARTESIAN_POINT ( 'NONE',  ( -24.92392925399193260, -294.4056183075323361, -346.3448827658697269 ) ) ;
#36629=CARTESIAN_POINT ( 'NONE',  ( -69.32173866297239329, -196.4524155619022565, -356.9615413897211624 ) ) ;
#36631=CARTESIAN_POINT ( 'NONE',  ( -97.41536935755578952, -271.8747392567533439, -222.9854645269756759 ) ) ;
#36632=CARTESIAN_POINT ( 'NONE',  ( -47.46423532620976005, -299.7827042058585789, -196.7672158356132286 ) ) ;
#36633=CARTESIAN_POINT ( 'NONE',  ( 34.49626605500665733, -289.0712801857098384, -285.9298822864070644 ) ) ;
#36635=CARTESIAN_POINT ( 'NONE',  ( -90.54034823450652425, -296.7245948484388691, -325.7761734532048763 ) ) ;
#36637=CARTESIAN_POINT ( 'NONE',  ( -91.57110656692699990, -285.7457798657515013, -221.3259721704485798 ) ) ;
#36638=CARTESIAN_POINT ( 'NONE',  ( -1.434003112007405933, -273.4373226177796710, -202.5958628330114664 ) ) ;
#36639=CARTESIAN_POINT ( 'NONE',  ( -13.82173177068103165, -295.5573199341579880, -343.5114420324887305 ) ) ;
#36640=CARTESIAN_POINT ( 'NONE',  ( 4.103099884259711061, -293.0865707134055356, -205.4762506825485104 ) ) ;
#36641=CARTESIAN_POINT ( 'NONE',  ( -28.10845212519906511, -292.3391532594212094, -197.8966477725577988 ) ) ;
#36643=CARTESIAN_POINT ( 'NONE',  ( -46.72683698870894631, -275.8540350931214675, -195.3862328366419661 ) ) ;
#36644=CARTESIAN_POINT ( 'NONE',  ( 38.98356100422601855, -274.4289974030442636, -276.8774997145287102 ) ) ;
#36646=VERTEX_POINT ( 'NONE', #70587 ) ;
#36647=CARTESIAN_POINT ( 'NONE',  ( -112.6560118505323231, -278.2574206360756079, -254.5724272502640133 ) ) ;
#36648=CARTESIAN_POINT ( 'NONE',  ( -2.518364395896292240, -272.9207702641687661, -205.2936475767278637 ) ) ;
#36649=CARTESIAN_POINT ( 'NONE',  ( -74.44163729380342431, -274.6262819062446852, -207.0739856390532907 ) ) ;
#36650=CARTESIAN_POINT ( 'NONE',  ( 33.73465197011300631, -276.2612301697394059, -252.7100380938230444 ) ) ;
#36651=CARTESIAN_POINT ( 'NONE',  ( -94.34139303504771590, -275.0017138394551353, -220.1116500895910235 ) ) ;
#36652=CARTESIAN_POINT ( 'NONE',  ( 37.10665934446651448, -273.7253860698702397, -282.3433314819762927 ) ) ;
#36653=CARTESIAN_POINT ( 'NONE',  ( -6.714656554497850038, -295.2905109197137676, -336.7378975856260013 ) ) ;
#36654=CARTESIAN_POINT ( 'NONE',  ( 26.29316446448969202, -292.6298897485842190, -307.3202700872212176 ) ) ;
#36656=CARTESIAN_POINT ( 'NONE',  ( -113.0039659906297231, -278.8689225160429146, -284.3886998550344742 ) ) ;
#36657=CARTESIAN_POINT ( 'NONE',  ( 25.27473730832239340, -275.2014886801561602, -232.7374641728282256 ) ) ;
#36659=CARTESIAN_POINT ( 'NONE',  ( -109.5065036537534979, -283.5595722876867057, -244.9536504930260605 ) ) ;
#36660=CARTESIAN_POINT ( 'NONE',  ( -110.5150792763383976, -298.3312968259965601, -287.6122056707797583 ) ) ;
#36663=CARTESIAN_POINT ( 'NONE',  ( -14.50591883633044787, -285.5529060375538961, -200.8016571277058802 ) ) ;
#36664=CARTESIAN_POINT ( 'NONE',  ( -91.72748636521008336, -276.0802501658214396, -320.6368910297986190 ) ) ;
#36665=CARTESIAN_POINT ( 'NONE',  ( -104.8188806823624759, -276.7337208366897698, -299.8522059376028892 ) ) ;
#36666=CARTESIAN_POINT ( 'NONE',  ( -99.83276915398350582, -285.9910701708554370, -311.9238242501832588 ) ) ;
#36667=CARTESIAN_POINT ( 'NONE',  ( 20.98779644816013601, -276.1338285978082467, -225.7893376335632070 ) ) ;
#36669=CARTESIAN_POINT ( 'NONE',  ( 18.30492762548804109, -274.6695298937160032, -322.4177528629518861 ) ) ;
#36670=CARTESIAN_POINT ( 'NONE',  ( 13.89264076929903702, -282.7684531189440804, -215.2893454459286886 ) ) ;
#36672=CARTESIAN_POINT ( 'NONE',  ( 27.67731376174091196, -289.9833601075466731, -308.8558192926971060 ) ) ;
#36673=CARTESIAN_POINT ( 'NONE',  ( 36.64245771789629202, -291.3901424460152612, -257.7559160641364997 ) ) ;
#36675=CARTESIAN_POINT ( 'NONE',  ( -106.7667882966642878, -271.5555031615079997, -246.2488677674949429 ) ) ;
#36676=CARTESIAN_POINT ( 'NONE',  ( -69.53214204160927636, -289.7635455518257572, -203.4543259998931717 ) ) ;
#36677=CARTESIAN_POINT ( 'NONE',  ( 69.94643833976951441, 44.42656045538938514, -317.4108715071801612 ) ) ;
#36678=CARTESIAN_POINT ( 'NONE',  ( -68.86555813957184569, -295.6375985272496791, -202.2938146962868871 ) ) ;
#36679=CARTESIAN_POINT ( 'NONE',  ( -9.831514472739019794, -287.1791487432359418, -341.5362360918209106 ) ) ;
#36680=CARTESIAN_POINT ( 'NONE',  ( -111.9983135034200075, -282.9748233684695720, -255.9327804085828575 ) ) ;
#36681=CARTESIAN_POINT ( 'NONE',  ( -89.29754886500192868, -285.2260625297558363, -322.5475412255105425 ) ) ;
#36682=CARTESIAN_POINT ( 'NONE',  ( -108.2472038397971090, -285.1175623923704165, -288.3891869536726063 ) ) ;
#36683=CARTESIAN_POINT ( 'NONE',  ( -68.65041975955305986, -291.4414453965063672, -338.9184353557639042 ) ) ;
#36684=AXIS2_PLACEMENT_3D ( 'NONE', #16737, #87756, #45131 ) ;
#36685=CARTESIAN_POINT ( 'NONE',  ( 11.76893841246079830, -275.0457258637568430, -211.0137858955411900 ) ) ;
#36687=CARTESIAN_POINT ( 'NONE',  ( 29.08487555839656125, -286.1080076658741405, -306.4819257647617405 ) ) ;
#36688=CARTESIAN_POINT ( 'NONE',  ( -72.84068338500294715, -277.5091989908727328, -338.7046018065634030 ) ) ;
#36689=CARTESIAN_POINT ( 'NONE',  ( 35.04719340458458987, -295.7671070719212025, -288.5736109239401799 ) ) ;
#36692=CARTESIAN_POINT ( 'NONE',  ( -74.05759101585547910, -282.2353711043031694, -334.0837607528757189 ) ) ;
#36694=CARTESIAN_POINT ( 'NONE',  ( -85.93000077804580883, -275.7228669243882564, -327.7808359982562934 ) ) ;
#36696=CARTESIAN_POINT ( 'NONE',  ( -89.67316056524549595, -271.8103758208579279, -214.7540714163802420 ) ) ;
#36697=CARTESIAN_POINT ( 'NONE',  ( 34.22283718884786197, -274.7034733493816816, -255.3865698946083853 ) ) ;
#36699=CARTESIAN_POINT ( 'NONE',  ( 34.31746227650188530, -294.8469177054485613, -253.1121476736348654 ) ) ;
#36700=CARTESIAN_POINT ( 'NONE',  ( 33.67716207303073617, -294.7286348754522010, -288.2421039859326584 ) ) ;
#36701=CARTESIAN_POINT ( 'NONE',  ( 23.49500095417907630, -294.3563020352347621, -224.1064653835943261 ) ) ;
#36702=CARTESIAN_POINT ( 'NONE',  ( 13.08346084051852820, -295.6803385282574368, -327.9691999329367036 ) ) ;
#36703=CARTESIAN_POINT ( 'NONE',  ( -107.8351052943669828, -296.6365429268314529, -251.3477277009112925 ) ) ;
#36704=CARTESIAN_POINT ( 'NONE',  ( -103.3927626519137419, -292.0794411334230176, -305.9994266604252857 ) ) ;
#36705=CARTESIAN_POINT ( 'NONE',  ( -104.4159720515098684, -284.2269055385384036, -308.2850021935161067 ) ) ;
#36706=CARTESIAN_POINT ( 'NONE',  ( -65.74186983552057484, -271.8242307191454188, -200.1066203008331001 ) ) ;
#36707=CARTESIAN_POINT ( 'NONE',  ( 39.35486919638645986, -287.2929035427188751, -262.9593731745756600 ) ) ;
#36708=CARTESIAN_POINT ( 'NONE',  ( -37.79500041815310851, -279.0377113513160907, -345.0172797319620486 ) ) ;
#36709=CARTESIAN_POINT ( 'NONE',  ( -103.8387429771259463, -283.7657820774043103, -239.1718336466684605 ) ) ;
#36710=CARTESIAN_POINT ( 'NONE',  ( 29.64716386366463041, -285.1064498332107746, -236.6343816037604881 ) ) ;
#36711=CARTESIAN_POINT ( 'NONE',  ( -81.49943007281909502, -277.5979657031264765, -208.7948905180417682 ) ) ;
#36712=CARTESIAN_POINT ( 'NONE',  ( -99.29329069375972949, -236.7418906163237580, -339.9611904871904358 ) ) ;
#36713=CARTESIAN_POINT ( 'NONE',  ( -108.4239255739651782, -284.2830928118351608, -253.4162636694933326 ) ) ;
#36714=CARTESIAN_POINT ( 'NONE',  ( 23.42291074594950118, -282.1315420025921412, -223.6956084102434090 ) ) ;
#36716=CARTESIAN_POINT ( 'NONE',  ( -67.97103996706708529, -288.5033034504162970, -340.7504904369728820 ) ) ;
#36717=CARTESIAN_POINT ( 'NONE',  ( -42.72905994652735018, -278.7191898495472628, -346.3704382653254470 ) ) ;
#36718=CARTESIAN_POINT ( 'NONE',  ( -9.376382623895057833, -278.0093201266830079, -341.5737523231353521 ) ) ;
#36719=CARTESIAN_POINT ( 'NONE',  ( -51.82528398430984140, -279.6950906817163514, -198.7606225066397201 ) ) ;
#36720=CARTESIAN_POINT ( 'NONE',  ( -27.08865172859196235, -276.1628889193509622, -196.3717911181254863 ) ) ;
#36721=CARTESIAN_POINT ( 'NONE',  ( 26.51174344813501449, -294.1191112121877040, -313.3929404336130347 ) ) ;
#36722=CARTESIAN_POINT ( 'NONE',  ( -2.623322973350376675, -286.6111685825279665, -336.4977058661108344 ) ) ;
#36723=CARTESIAN_POINT ( 'NONE',  ( -103.9209820452293513, -292.6377788681243715, -233.2984732700124653 ) ) ;
#36724=CARTESIAN_POINT ( 'NONE',  ( -45.13721603296350082, -294.0733770383077967, -343.3052652123174653 ) ) ;
#36725=CARTESIAN_POINT ( 'NONE',  ( 17.98567555085146097, -293.8975469755371819, -318.0348663922093806 ) ) ;
#36726=CARTESIAN_POINT ( 'NONE',  ( -70.77542480646489764, -292.7010869421544612, -201.3417108164417186 ) ) ;
#36727=CARTESIAN_POINT ( 'NONE',  ( 20.59163003303796913, -281.5767518879754334, -225.7580228462045113 ) ) ;
#36728=CARTESIAN_POINT ( 'NONE',  ( -36.88527894149524400, -296.9780751899973552, -193.6703088412876923 ) ) ;
#36729=CARTESIAN_POINT ( 'NONE',  ( -12.24914102296441420, -289.3856352070126263, -343.1058186220211041 ) ) ;
#36730=CARTESIAN_POINT ( 'NONE',  ( -98.80063803479879425, -282.0937129488573305, -314.7557629154503616 ) ) ;
#36731=CARTESIAN_POINT ( 'NONE',  ( 20.55979956657802177, -288.5720723814009148, -321.1073080936008068 ) ) ;
#36732=CARTESIAN_POINT ( 'NONE',  ( -83.66455760767969707, -285.7296347783826036, -213.8482704037640758 ) ) ;
#36733=CARTESIAN_POINT ( 'NONE',  ( 197.0526034356786909, 285.3763918475410719, -111.7597976791601440 ) ) ;
#36734=CARTESIAN_POINT ( 'NONE',  ( -57.42940174176641932, -168.5846715610379931, -362.5153972683089592 ) ) ;
#36735=CARTESIAN_POINT ( 'NONE',  ( 179.1287263462807573, 251.3206971305780257, -164.1895290402175362 ) ) ;
#36736=CARTESIAN_POINT ( 'NONE',  ( -92.32304736588534411, -278.4369178665999698, -222.0755825259350331 ) ) ;
#36737=CARTESIAN_POINT ( 'NONE',  ( 15.49165899291676141, -279.7411057749791325, -219.4667166436613570 ) ) ;
#36738=CARTESIAN_POINT ( 'NONE',  ( 23.61869896377583444, -274.5911370579396475, -223.3335545625459702 ) ) ;
#36739=CARTESIAN_POINT ( 'NONE',  ( -110.3740896168006174, -272.9989044831370961, -270.3668062096999734 ) ) ;
#36740=CARTESIAN_POINT ( 'NONE',  ( -81.88057515096950567, -278.0330392942730668, -208.2733180284720618 ) ) ;
#36741=CARTESIAN_POINT ( 'NONE',  ( -45.85146970287838286, -281.1805351109912863, -344.5714084857896182 ) ) ;
#36742=CARTESIAN_POINT ( 'NONE',  ( -69.08391957842276554, -297.2240279907319405, -339.4145181524082204 ) ) ;
#36743=CARTESIAN_POINT ( 'NONE',  ( -34.86146857238223618, -292.5764957798779164, -197.3416897922132023 ) ) ;
#36744=CARTESIAN_POINT ( 'NONE',  ( -78.46413158314939551, -288.3029789028551022, -331.3337140688640829 ) ) ;
#36745=CARTESIAN_POINT ( 'NONE',  ( -7.737501600269742319, -275.0813584043654032, -199.3334482253517024 ) ) ;
#36746=CARTESIAN_POINT ( 'NONE',  ( -108.7795722901818181, -296.9177619382888906, -255.2800064297944687 ) ) ;
#36750=CARTESIAN_POINT ( 'NONE',  ( -103.5439180514777746, -280.9530209141566388, -233.9388646535291230 ) ) ;
#36751=CIRCLE ( 'NONE', #54927, 2.939656322713313230 ) ;
#36753=CARTESIAN_POINT ( 'NONE',  ( 20.75249025025642169, -282.0049406448960099, -225.6272876952578770 ) ) ;
#36754=CARTESIAN_POINT ( 'NONE',  ( -99.43405333055756046, -280.8995585493619842, -226.5602767991605333 ) ) ;
#36755=CARTESIAN_POINT ( 'NONE',  ( 12.06662934367147244, -281.4032824717512540, -324.4187300865832526 ) ) ;
#36756=CARTESIAN_POINT ( 'NONE',  ( -74.60743724592036585, -272.0269079481059862, -206.7255040913486255 ) ) ;
#36760=CARTESIAN_POINT ( 'NONE',  ( 39.15551659369661763, -276.2575460780564640, -262.5864954224175563 ) ) ;
#36762=CARTESIAN_POINT ( 'NONE',  ( 22.03347999966414150, -276.9242011569562010, -224.5189540467830511 ) ) ;
#36763=CARTESIAN_POINT ( 'NONE',  ( -71.32522730692068080, -276.0668272448311882, -338.7988720054276541 ) ) ;
#36766=CARTESIAN_POINT ( 'NONE',  ( -102.9718258805812781, -286.0398257718971990, -307.4950212589780563 ) ) ;
#36768=CARTESIAN_POINT ( 'NONE',  ( -89.92528967113392468, -290.4827866808067824, -219.4929763052819567 ) ) ;
#36769=CARTESIAN_POINT ( 'NONE',  ( 35.75473705710635386, -286.5979917014230409, -246.3114117091276398 ) ) ;
#36770=CARTESIAN_POINT ( 'NONE',  ( -36.20007475029898814, -281.2775027747325112, -344.3656496525327384 ) ) ;
#36771=CARTESIAN_POINT ( 'NONE',  ( -69.28119369061114696, -282.0555552826351118, -336.6716682828496801 ) ) ;
#36772=CARTESIAN_POINT ( 'NONE',  ( 7.819583032856252558, -284.7537931863032554, -211.1201959393978029 ) ) ;
#36773=CARTESIAN_POINT ( 'NONE',  ( 34.62302802845156435, -282.9473799628081565, -284.8538604442662745 ) ) ;
#36774=CARTESIAN_POINT ( 'NONE',  ( 31.87779560526152167, -273.1734711437652550, -241.3536662796325913 ) ) ;
#36775=CARTESIAN_POINT ( 'NONE',  ( -65.56194681057962725, -284.0891331744151671, -199.5653484693689848 ) ) ;
#36776=CARTESIAN_POINT ( 'NONE',  ( -112.3117419303367654, -298.5973368378957957, -266.8548584266072226 ) ) ;
#36778=CARTESIAN_POINT ( 'NONE',  ( -108.0442996236418622, -279.2420133269375810, -289.4543333536269643 ) ) ;
#36779=CARTESIAN_POINT ( 'NONE',  ( -112.3764240251258855, -286.4849981587564116, -275.6156172564502640 ) ) ;
#36782=CARTESIAN_POINT ( 'NONE',  ( 36.06695296336238954, -295.7011276235264177, -288.3173934333239004 ) ) ;
#36784=CARTESIAN_POINT ( 'NONE',  ( -75.04000715050869985, -275.5542320894206796, -335.1981313066179951 ) ) ;
#36785=CARTESIAN_POINT ( 'NONE',  ( -8.303650606907879705, -287.8786717017288765, -341.5157111399344103 ) ) ;
#36786=CARTESIAN_POINT ( 'NONE',  ( 21.64537437584522550, -291.3360073274541264, -226.0106336735533716 ) ) ;
#36787=CARTESIAN_POINT ( 'NONE',  ( -45.98259260431741779, -275.8486937439034250, -343.3954984292109884 ) ) ;
#36788=CARTESIAN_POINT ( 'NONE',  ( -85.29374223801329435, -293.8620258123667668, -327.0984375345110493 ) ) ;
#36789=CARTESIAN_POINT ( 'NONE',  ( -49.78861539303773043, -293.2053837619742467, -197.8779746303997058 ) ) ;
#36790=CARTESIAN_POINT ( 'NONE',  ( -85.33152481854862970, -275.9090924074130839, -210.2361428286348826 ) ) ;
#36792=CARTESIAN_POINT ( 'NONE',  ( -25.03884946062321504, -293.3780089964228637, -345.7230450274479381 ) ) ;
#36793=CARTESIAN_POINT ( 'NONE',  ( 34.48434176199818779, -289.3735293157934052, -287.3157670210113110 ) ) ;
#36794=CARTESIAN_POINT ( 'NONE',  ( -109.8221491066610866, -288.4995110242126657, -293.3489331880157920 ) ) ;
#36795=CARTESIAN_POINT ( 'NONE',  ( 18.28274548461518734, -289.6591956413274147, -318.6172661711337355 ) ) ;
#36797=CARTESIAN_POINT ( 'NONE',  ( -71.23851263373516929, -290.3144726487295202, -335.2105069138991666 ) ) ;
#36799=CARTESIAN_POINT ( 'NONE',  ( 19.34082124355152743, -289.4612870093533843, -321.9083279324900104 ) ) ;
#36800=CARTESIAN_POINT ( 'NONE',  ( -104.6939055459116759, -277.0178205906348694, -236.4501987292175045 ) ) ;
#36801=CARTESIAN_POINT ( 'NONE',  ( -62.04486340233327013, -280.0729714785089755, -197.3974378045095364 ) ) ;
#36802=CARTESIAN_POINT ( 'NONE',  ( 37.96486863945008849, -281.0184492793648019, -254.3398145777974264 ) ) ;
#36803=CARTESIAN_POINT ( 'NONE',  ( 16.48206017951068958, -284.8170321380278551, -218.1308252914413686 ) ) ;
#36804=CARTESIAN_POINT ( 'NONE',  ( -112.3417001281054297, -274.5519904173220311, -270.3865538441530134 ) ) ;
#36805=CARTESIAN_POINT ( 'NONE',  ( -67.79164321634486612, -277.7878204436214560, -202.6445037518199399 ) ) ;
#36807=CARTESIAN_POINT ( 'NONE',  ( -37.34053867939269367, -281.0519445936344027, -345.3738477710438133 ) ) ;
#36808=CARTESIAN_POINT ( 'NONE',  ( 197.1939413472297531, 281.6276417382965178, -110.3312367469949464 ) ) ;
#36809=CARTESIAN_POINT ( 'NONE',  ( -92.84312659188438488, -276.3098641460309750, -322.8039304740246962 ) ) ;
#36810=CARTESIAN_POINT ( 'NONE',  ( -102.2495113585714250, -284.0095371113371812, -229.5142264162927006 ) ) ;
#36811=CARTESIAN_POINT ( 'NONE',  ( -54.25877517958490159, -274.6320935663379714, -199.1823690604259411 ) ) ;
#36812=CARTESIAN_POINT ( 'NONE',  ( -93.17494621273786493, -292.8324584107060105, -222.1004813491875893 ) ) ;
#36813=CARTESIAN_POINT ( 'NONE',  ( 30.22961323696181068, -300.1966590518934481, -193.8395018425161709 ) ) ;
#36814=CARTESIAN_POINT ( 'NONE',  ( 25.29614986399421284, -274.7016079911401789, -232.7320200206928007 ) ) ;
#36815=CARTESIAN_POINT ( 'NONE',  ( 7.272559309870788802, -296.4447451376365166, -330.7132379572404943 ) ) ;
#36816=CARTESIAN_POINT ( 'NONE',  ( -8.231165223220649807, -288.8480277823040865, -341.6605635237885963 ) ) ;
#36818=CARTESIAN_POINT ( 'NONE',  ( 12.06932601694004248, -278.8129495320926594, -213.1958777518001682 ) ) ;
#36819=CARTESIAN_POINT ( 'NONE',  ( -37.79290030657497113, -291.8799680262281413, -193.3624399228993411 ) ) ;
#36820=CARTESIAN_POINT ( 'NONE',  ( -109.1718583294079679, -289.4223191808246156, -284.7024570135646400 ) ) ;
#36823=CARTESIAN_POINT ( 'NONE',  ( 26.39254997012500326, -292.0839678361840015, -309.9927494513522674 ) ) ;
#36827=CARTESIAN_POINT ( 'NONE',  ( -107.0126802088411182, -289.7664392164821265, -292.5272007342535403 ) ) ;
#36829=CARTESIAN_POINT ( 'NONE',  ( 18.17302546201613467, -287.7654569333693075, -217.2662141498794028 ) ) ;
#36830=CARTESIAN_POINT ( 'NONE',  ( -53.35057174420112602, -294.3376638359845288, -200.3683826091709648 ) ) ;
#36831=CARTESIAN_POINT ( 'NONE',  ( -44.78477869464024508, -294.2027940696279416, -346.8173774530810078 ) ) ;
#36832=CARTESIAN_POINT ( 'NONE',  ( -34.48053704472732051, -284.3320607180696129, -346.8144502818275896 ) ) ;
#36833=CARTESIAN_POINT ( 'NONE',  ( -72.37214735263843579, -285.4082075762343038, -206.3010760867753390 ) ) ;
#36835=CARTESIAN_POINT ( 'NONE',  ( 0.8545650129210551338, -275.8885338214997773, -207.5734694588424247 ) ) ;
#36836=CARTESIAN_POINT ( 'NONE',  ( -20.50106539893686275, -292.8550685056684415, -343.1346769554493790 ) ) ;
#36838=CARTESIAN_POINT ( 'NONE',  ( 35.23659445264143386, -274.2025218373474900, -259.3438418468474538 ) ) ;
#36841=CARTESIAN_POINT ( 'NONE',  ( -65.59968739739146315, -295.0784319070454558, -341.9800181438119466 ) ) ;
#36842=CARTESIAN_POINT ( 'NONE',  ( -52.40372891949215273, -287.7779160959167370, -197.4608471762732904 ) ) ;
#36843=AXIS2_PLACEMENT_3D ( 'NONE', #29822, #42607, #71522 ) ;
#36844=CARTESIAN_POINT ( 'NONE',  ( -107.4958552754885943, -298.0301750027059029, -239.2477230367415757 ) ) ;
#36845=CARTESIAN_POINT ( 'NONE',  ( 33.80760680919627248, -287.9817675162150294, -253.5240536369941537 ) ) ;
#36846=CARTESIAN_POINT ( 'NONE',  ( -80.10508841278016234, -276.6740518776620661, -334.1755084955324264 ) ) ;
#36847=CARTESIAN_POINT ( 'NONE',  ( 4.179250514901015734, -295.1600395455890862, -335.1487979821375234 ) ) ;
#36848=CARTESIAN_POINT ( 'NONE',  ( -96.34334640992992149, -288.0440245773420429, -317.9116936895005097 ) ) ;
#36849=CARTESIAN_POINT ( 'NONE',  ( 6.605412711137148563, -294.8062076753766974, -333.6273014008230007 ) ) ;
#36850=CARTESIAN_POINT ( 'NONE',  ( -32.16002058906382643, -292.4525599200878219, -197.5114314398128101 ) ) ;
#36854=CARTESIAN_POINT ( 'NONE',  ( 174.1105135456032542, 240.3386868885705496, -177.2113801462826643 ) ) ;
#36855=CARTESIAN_POINT ( 'NONE',  ( 33.21091871336700052, -288.6979250818966420, -241.1536667946379566 ) ) ;
#36856=CARTESIAN_POINT ( 'NONE',  ( -111.2586520408596868, -282.4809262143061233, -234.7283546768995564 ) ) ;
#36858=CARTESIAN_POINT ( 'NONE',  ( -14.25045192895701263, -279.6923947753392099, -196.9560768477662123 ) ) ;
#36859=CARTESIAN_POINT ( 'NONE',  ( -43.04791768223248738, -285.1243805308062633, -345.0279269821415937 ) ) ;
#36860=CARTESIAN_POINT ( 'NONE',  ( -49.23497188951420611, -284.4782885979726075, -194.8282850317589237 ) ) ;
#36861=CARTESIAN_POINT ( 'NONE',  ( -70.63810939896589502, -287.5745296107767786, -336.9535029898096354 ) ) ;
#36862=CARTESIAN_POINT ( 'NONE',  ( 22.64019871995547462, -276.7844792345271685, -224.0531067116369570 ) ) ;
#36864=CARTESIAN_POINT ( 'NONE',  ( -44.58141681695952485, -298.4505642652458732, -197.6087337851072334 ) ) ;
#36865=CARTESIAN_POINT ( 'NONE',  ( -39.72167468022215076, -293.7674540402812795, -343.8282385825488063 ) ) ;
#36866=CARTESIAN_POINT ( 'NONE',  ( -86.74559198605830090, -280.0376532944069368, -211.3632058533457894 ) ) ;
#36867=CARTESIAN_POINT ( 'NONE',  ( 34.70715861495462207, -275.7111269127703395, -282.4122724066306773 ) ) ;
#36868=CARTESIAN_POINT ( 'NONE',  ( -110.0666238457801853, -278.0047955269531030, -262.4617719167286509 ) ) ;
#36869=CARTESIAN_POINT ( 'NONE',  ( -24.22605246357979780, -275.2953893996891566, -194.7461205898380854 ) ) ;
#36870=CARTESIAN_POINT ( 'NONE',  ( -4.141159238860603331, -275.5449661269385615, -339.5074353515473149 ) ) ;
#36871=CARTESIAN_POINT ( 'NONE',  ( 153.3814170967218615, 207.2574094406980976, -217.2232996820281130 ) ) ;
#36872=CARTESIAN_POINT ( 'NONE',  ( -59.62836778256614423, -275.3404975800690977, -342.0270585912988395 ) ) ;
#36873=CARTESIAN_POINT ( 'NONE',  ( -113.3551985198493668, -297.8793511262754237, -278.1427858135329529 ) ) ;
#36874=CARTESIAN_POINT ( 'NONE',  ( 10.64812456238590066, -278.9090924074130839, -330.4860931364851808 ) ) ;
#36875=CARTESIAN_POINT ( 'NONE',  ( -69.18520112214993389, -196.4157418647702968, -356.4528236438462159 ) ) ;
#36876=CARTESIAN_POINT ( 'NONE',  ( -33.23503331000667060, -287.1846106216869998, -197.1170884104619461 ) ) ;
#36877=CARTESIAN_POINT ( 'NONE',  ( -35.19956408150198257, -287.8388036625057111, -194.3916777255585941 ) ) ;
#36878=CARTESIAN_POINT ( 'NONE',  ( -38.61837901735849954, -285.3843446657514278, -197.2578343958313667 ) ) ;
#36879=CARTESIAN_POINT ( 'NONE',  ( -99.86356443370645763, -276.4153224812768030, -309.6670332139806874 ) ) ;
#36880=CARTESIAN_POINT ( 'NONE',  ( -100.6752999083492739, -286.9384364619213557, -231.5369026772743837 ) ) ;
#36881=CARTESIAN_POINT ( 'NONE',  ( -109.2793814135444421, -277.2416644144022939, -254.3134942990032528 ) ) ;
#36882=CARTESIAN_POINT ( 'NONE',  ( -1.213292271919899745, -277.8776866301691939, -334.4185682969979894 ) ) ;
#36883=CARTESIAN_POINT ( 'NONE',  ( 35.66376543588182813, -276.0965471303533718, -274.3097109336476365 ) ) ;
#36884=CARTESIAN_POINT ( 'NONE',  ( 36.75640753453114229, -286.5915451010758375, -289.7899409132114101 ) ) ;
#36885=CARTESIAN_POINT ( 'NONE',  ( 39.45873257429219905, -282.3853018712736116, -272.7802824541742552 ) ) ;
#36886=CARTESIAN_POINT ( 'NONE',  ( 38.81125129804725304, -282.1817532547462974, -281.3271971504478302 ) ) ;
#36890=CARTESIAN_POINT ( 'NONE',  ( 18.72638111791853177, -290.1165214094963289, -321.3380371559483137 ) ) ;
#36891=CARTESIAN_POINT ( 'NONE',  ( -106.8056060178617344, -289.6512339624493961, -238.1715188204582603 ) ) ;
#36892=CARTESIAN_POINT ( 'NONE',  ( -67.14230893970606928, -272.7103626360679982, -203.4494586486582932 ) ) ;
#36893=CARTESIAN_POINT ( 'NONE',  ( 6.445004935181720462, -291.9787336868825491, -207.1469008630812141 ) ) ;
#36894=CARTESIAN_POINT ( 'NONE',  ( 20.06739938321959116, -285.3847274916469701, -224.1361075000812377 ) ) ;
#36895=CARTESIAN_POINT ( 'NONE',  ( 35.52023449991650494, -288.8733082969592942, -279.2080941264615035 ) ) ;
#36896=CARTESIAN_POINT ( 'NONE',  ( -85.33152481854864391, -299.9090924074131408, -210.2361428286349110 ) ) ;
#36898=CARTESIAN_POINT ( 'NONE',  ( -41.62032255882137122, -291.1061843189511933, -345.2518576254083769 ) ) ;
#36899=CARTESIAN_POINT ( 'NONE',  ( -108.1473928269375193, -288.2239917012337287, -295.7461585387530931 ) ) ;
#36900=CARTESIAN_POINT ( 'NONE',  ( -9.649097243101797616, -290.6905552127029750, -340.0750330642770791 ) ) ;
#36901=CARTESIAN_POINT ( 'NONE',  ( -94.46102003390205937, -284.8475454532908202, -316.2154575172493765 ) ) ;
#36902=CARTESIAN_POINT ( 'NONE',  ( -111.1302534931136705, -292.7367265589002159, -255.9664317823821023 ) ) ;
#36903=CARTESIAN_POINT ( 'NONE',  ( 82.13382245134783943, -300.7353340821118195, -193.7454283942308280 ) ) ;
#36905=VECTOR ( 'NONE', #72898, 1000.000000000000000 ) ;
#36906=CARTESIAN_POINT ( 'NONE',  ( -29.27652873796473187, -300.0725136216683495, -194.7984956000887280 ) ) ;
#36907=CARTESIAN_POINT ( 'NONE',  ( -26.72943433756234910, -282.1110169046190208, -342.8002470040619869 ) ) ;
#36908=CARTESIAN_POINT ( 'NONE',  ( -94.08863254628134598, -281.8717741505666368, -319.4192907530908769 ) ) ;
#36909=CARTESIAN_POINT ( 'NONE',  ( 8.801014963468832164, -293.6344376790679007, -331.8022171262888946 ) ) ;
#36910=CARTESIAN_POINT ( 'NONE',  ( -104.1097020931474617, -271.2180401522759894, -238.4235550751121764 ) ) ;
#36911=CARTESIAN_POINT ( 'NONE',  ( 29.30914618979764441, -274.0741951566227499, -303.6280945954125059 ) ) ;
#36912=CARTESIAN_POINT ( 'NONE',  ( -80.02799379651372647, -298.7759356325807403, -210.5353391772223119 ) ) ;
#36915=CARTESIAN_POINT ( 'NONE',  ( -105.5931858780995896, -295.2266800366576263, -236.9588919460001932 ) ) ;
#36917=CARTESIAN_POINT ( 'NONE',  ( 20.16551058940973817, -295.6210030010713012, -316.2973931938221313 ) ) ;
#36920=CARTESIAN_POINT ( 'NONE',  ( -63.61746002073931550, -296.2063128363726037, -338.6949943381572439 ) ) ;
#36922=CARTESIAN_POINT ( 'NONE',  ( -94.55095229357320363, -283.2492345915375154, -221.2369024467940903 ) ) ;
#36923=CARTESIAN_POINT ( 'NONE',  ( -104.9619019494661245, -296.1837140179526386, -297.8658140476903782 ) ) ;
#36925=CARTESIAN_POINT ( 'NONE',  ( -111.4914709271562003, -284.2920650769411282, -291.1171168851585662 ) ) ;
#36926=CARTESIAN_POINT ( 'NONE',  ( 16.81163618459275000, -284.2091697568932318, -323.1305958465078447 ) ) ;
#36927=CARTESIAN_POINT ( 'NONE',  ( 24.68875090346103462, -286.6132069863242009, -224.7763898775358200 ) ) ;
#36928=CARTESIAN_POINT ( 'NONE',  ( -44.44960301515508405, -289.9619948487066381, -195.8140171833827878 ) ) ;
#36929=CARTESIAN_POINT ( 'NONE',  ( -14.26648824407761396, -279.5409997918751515, -197.0134952603672218 ) ) ;
#36930=CARTESIAN_POINT ( 'NONE',  ( 31.95455697924147387, -273.4809262143061233, -303.7686719486574134 ) ) ;
#36932=CARTESIAN_POINT ( 'NONE',  ( 22.32328254390262501, -285.7518421287712158, -227.5294096280811686 ) ) ;
#36933=CARTESIAN_POINT ( 'NONE',  ( -102.0478770743834929, -288.9296200951868627, -311.6244275673911943 ) ) ;
#36935=CARTESIAN_POINT ( 'NONE',  ( -96.58593854714524696, -279.3246251290308919, -318.6384823448831867 ) ) ;
#36936=CARTESIAN_POINT ( 'NONE',  ( -65.02326372284356637, -293.4320866481708094, -340.4616835367447152 ) ) ;
#36937=CARTESIAN_POINT ( 'NONE',  ( 35.58682598292216426, -281.2673555978400373, -274.0377422451885536 ) ) ;
#36938=CARTESIAN_POINT ( 'NONE',  ( -24.90572107143746550, -295.0645394442873908, -346.4043043483591759 ) ) ;
#36939=CARTESIAN_POINT ( 'NONE',  ( 6.724355481774723309, -284.7256879460035748, -208.9167217821592430 ) ) ;
#36941=CARTESIAN_POINT ( 'NONE',  ( -69.13826660988181061, -281.6341555427423486, -202.4208243649676717 ) ) ;
#36942=CARTESIAN_POINT ( 'NONE',  ( -110.2835078175194070, -295.7042042218030815, -263.2649739798760038 ) ) ;
#36945=CARTESIAN_POINT ( 'NONE',  ( 34.30644308138853660, -283.2611589842876469, -249.4233440177841601 ) ) ;
#36946=DIRECTION ( 'NONE',  ( 0.9951408606192333473, 0.000000000000000000, -0.09846150276129089773 ) ) ;
#36947=CARTESIAN_POINT ( 'NONE',  ( -82.08285599513421005, -294.9094976428775681, -214.2051214447836571 ) ) ;
#36948=CARTESIAN_POINT ( 'NONE',  ( 22.63873250808064341, -274.1044569133171080, -222.3141468171702684 ) ) ;
#36949=CARTESIAN_POINT ( 'NONE',  ( -109.6232494068969316, -290.2495149318017980, -280.6673531531192793 ) ) ;
#36950=CARTESIAN_POINT ( 'NONE',  ( 14.42537766125526488, -283.8284502065166066, -322.8817930029990748 ) ) ;
#36951=CARTESIAN_POINT ( 'NONE',  ( -24.47679064279848404, -275.8190786879782195, -197.6389279314454654 ) ) ;
#36952=CARTESIAN_POINT ( 'NONE',  ( 6.481749951803364773, -284.0681167762502355, -332.7630064512111971 ) ) ;
#36953=CARTESIAN_POINT ( 'NONE',  ( 34.32482175247959333, -280.5549554248458435, -286.2053645005437943 ) ) ;
#36955=CARTESIAN_POINT ( 'NONE',  ( -3.824187849458207555, -274.3154723379626603, -201.0243446290846521 ) ) ;
#36956=CARTESIAN_POINT ( 'NONE',  ( 36.97054912080180600, -295.4054481140806843, -265.1924673239111030 ) ) ;
#36957=DIRECTION ( 'NONE',  ( 0.000000000000000000, 0.000000000000000000, 1.000000000000000000 ) ) ;
#36958=DIRECTION ( 'NONE',  ( 1.000000000000000000, 0.000000000000000000, 0.000000000000000000 ) ) ;
#36959=CARTESIAN_POINT ( 'NONE',  ( 5.889451509615496683, -292.6128637411753743, -332.6453887780560876 ) ) ;
#36960=CARTESIAN_POINT ( 'NONE',  ( -92.95655378125168511, -272.7333711148331190, -222.9606251350134301 ) ) ;
#36962=CARTESIAN_POINT ( 'NONE',  ( -83.85915103086674094, -292.9469145962386278, -209.8062095858481655 ) ) ;
#36963=CARTESIAN_POINT ( 'NONE',  ( -106.6662871844225293, -281.4805209788417528, -237.0123917617630980 ) ) ;
#36964=CARTESIAN_POINT ( 'NONE',  ( 26.15512029855018383, -294.1886004579299083, -227.4173669537807712 ) ) ;
#36965=CARTESIAN_POINT ( 'NONE',  ( -79.17879856468479716, -291.6177795230280481, -332.4693228246752597 ) ) ;
#36966=CARTESIAN_POINT ( 'NONE',  ( -37.84707834972281404, -275.0583030169848371, -345.2055143726373103 ) ) ;
#36967=CARTESIAN_POINT ( 'NONE',  ( -94.70027095998874245, -279.8124312193276069, -317.8290373671133580 ) ) ;
#36968=CARTESIAN_POINT ( 'NONE',  ( -2.490811265811056607, -292.6672015917673662, -336.1389998699629587 ) ) ;
#36969=CARTESIAN_POINT ( 'NONE',  ( 27.26432475088252616, -283.9392126661333009, -310.0379450181517313 ) ) ;
#36971=CARTESIAN_POINT ( 'NONE',  ( -95.13577766700244354, -283.5904542133199584, -315.0125967312922057 ) ) ;
#36972=CARTESIAN_POINT ( 'NONE',  ( 5.998200796796139045, -281.7048132604465422, -207.0907023297529008 ) ) ;
#36973=CARTESIAN_POINT ( 'NONE',  ( 34.21111404242772380, -280.6951801885720101, -297.7144267780789733 ) ) ;
#36975=CARTESIAN_POINT ( 'NONE',  ( 10.38916068597229803, -277.3531791362818808, -330.5504237604178570 ) ) ;
#36977=CARTESIAN_POINT ( 'NONE',  ( 36.22242171068192818, -277.3291043189938136, -290.6837035835468441 ) ) ;
#36978=CARTESIAN_POINT ( 'NONE',  ( -67.68488546085839630, -285.9805209788416391, -333.4427485647536855 ) ) ;
#36979=ORIENTED_EDGE ( 'NONE', *, *, #72569, .F. ) ;
#36980=CARTESIAN_POINT ( 'NONE',  ( -112.1750334612141984, -274.5519907627465273, -270.3865268295556348 ) ) ;
#36981=CARTESIAN_POINT ( 'NONE',  ( -102.0203561698286876, -276.0713964293829008, -307.7278154579086049 ) ) ;
#36982=CARTESIAN_POINT ( 'NONE',  ( -95.81366283558585906, -292.9736842513708552, -221.8126232103016946 ) ) ;
#36983=CARTESIAN_POINT ( 'NONE',  ( -75.02505197771870371, -290.8847456637496407, -207.6613210053333205 ) ) ;
#36984=CARTESIAN_POINT ( 'NONE',  ( 35.01245512179372099, -287.3922101514290262, -296.6771863954621722 ) ) ;
#36986=CARTESIAN_POINT ( 'NONE',  ( 36.14253679120695750, -291.8617747428961593, -249.3688743060224908 ) ) ;
#36987=CARTESIAN_POINT ( 'NONE',  ( -105.3266632753537522, -283.3347995887914976, -241.5160031345323262 ) ) ;
#36988=CARTESIAN_POINT ( 'NONE',  ( -109.3117356732567629, -292.6493620579727803, -252.1110151878432362 ) ) ;
#36989=CARTESIAN_POINT ( 'NONE',  ( -104.1054789661079951, -283.4507865373743698, -239.0423711642947922 ) ) ;
#36990=CARTESIAN_POINT ( 'NONE',  ( 27.29668544199265767, -283.3412964415218198, -305.3342875222486441 ) ) ;
#36991=CARTESIAN_POINT ( 'NONE',  ( -107.5114081177776910, -291.0934486694390557, -301.6210938016452019 ) ) ;
#36992=CARTESIAN_POINT ( 'NONE',  ( -4.325365113249699967, -280.9918637714453098, -205.1712226753450921 ) ) ;
#36993=CARTESIAN_POINT ( 'NONE',  ( 31.83402857222822391, -291.9217358041721582, -237.3329715404935598 ) ) ;
#36994=CIRCLE ( 'NONE', #26449, 2.738891987356051327 ) ;
#36995=CARTESIAN_POINT ( 'NONE',  ( 39.41572584169161075, -288.2980425069398507, -265.8177318945975003 ) ) ;
#36996=CARTESIAN_POINT ( 'NONE',  ( 24.09685428922209738, -288.6616747870603490, -316.6734374510982093 ) ) ;
#36997=CARTESIAN_POINT ( 'NONE',  ( -2.188249144733531715, -286.6975704660616771, -206.3260084878871226 ) ) ;
#37000=CARTESIAN_POINT ( 'NONE',  ( 38.47554935220361472, -295.4116289293041859, -270.2871325723973541 ) ) ;
#37001=CARTESIAN_POINT ( 'NONE',  ( -36.29808382088275920, -293.7241940474278294, -346.8738709653217143 ) ) ;
#37002=CARTESIAN_POINT ( 'NONE',  ( -108.7182843014649336, -277.3945864456988488, -286.8116003028404748 ) ) ;
#37003=CARTESIAN_POINT ( 'NONE',  ( -87.38962092380074864, -296.7242667153077491, -211.9084106621063484 ) ) ;
#37004=CARTESIAN_POINT ( 'NONE',  ( 33.98410035876713664, -291.7897037976191541, -251.8317375574839048 ) ) ;
#37005=CARTESIAN_POINT ( 'NONE',  ( -8.597701657243348450, -276.1935715257366155, -202.1026798337757100 ) ) ;
#37006=CARTESIAN_POINT ( 'NONE',  ( -104.6306431716327552, -295.2035005546922548, -239.4129797224479148 ) ) ;
#37007=CARTESIAN_POINT ( 'NONE',  ( 26.57282121197138380, -294.2647322262678813, -234.1732512066087111 ) ) ;
#37008=CARTESIAN_POINT ( 'NONE',  ( 30.87824537295921701, -294.9908543258464988, -297.3378299978240307 ) ) ;
#37010=CARTESIAN_POINT ( 'NONE',  ( 27.96881088667049298, -292.0482342388298775, -307.6759528381567179 ) ) ;
#37011=CARTESIAN_POINT ( 'NONE',  ( -53.44865136905574587, -290.2051414032908951, -341.8032243980975977 ) ) ;
#37012=CARTESIAN_POINT ( 'NONE',  ( -12.99719401820812870, -295.0603300179528219, -339.2579291907965171 ) ) ;
#37013=CARTESIAN_POINT ( 'NONE',  ( -109.7636072712097217, -280.7987700860118707, -249.5410754765287891 ) ) ;
#37014=CARTESIAN_POINT ( 'NONE',  ( -112.2313437181619662, -277.4347271936559309, -254.6506584485609324 ) ) ;
#37015=CARTESIAN_POINT ( 'NONE',  ( 9.454885671036437955, -274.0253381202152809, -209.3415117578530840 ) ) ;
#37016=CARTESIAN_POINT ( 'NONE',  ( -70.88528326492306064, -281.5780024296843749, -336.8294352962802805 ) ) ;
#37017=CARTESIAN_POINT ( 'NONE',  ( -113.2450508922976695, -277.0441683364643382, -263.0699910422949301 ) ) ;
#37018=CARTESIAN_POINT ( 'NONE',  ( -28.41678812943368371, -278.1648302364130814, -195.6738277291115367 ) ) ;
#37020=CARTESIAN_POINT ( 'NONE',  ( -98.32135777670937671, -271.6959551582586982, -229.0773264192933425 ) ) ;
#37021=CARTESIAN_POINT ( 'NONE',  ( 27.60217406688886399, -277.0503887539096013, -232.7446843780067809 ) ) ;
#37023=CARTESIAN_POINT ( 'NONE',  ( -91.60967520620930316, -289.3043573793663654, -218.0050431614291711 ) ) ;
#37024=CARTESIAN_POINT ( 'NONE',  ( -112.6399703681933602, -290.7542311198969855, -254.2001374818672161 ) ) ;
#37025=CARTESIAN_POINT ( 'NONE',  ( -41.12656548946259960, -276.0049114333808689, -195.2387825725652988 ) ) ;
#37026=CARTESIAN_POINT ( 'NONE',  ( -92.57874459094192332, -271.2609296130669918, -219.6087962519301300 ) ) ;
#37027=CARTESIAN_POINT ( 'NONE',  ( -109.1556968857388341, -283.4009858888555868, -297.8390650868544185 ) ) ;
#37029=CARTESIAN_POINT ( 'NONE',  ( -28.31812375890616096, -280.9376230016517866, -344.8679413759246586 ) ) ;
#37031=CARTESIAN_POINT ( 'NONE',  ( -38.89065619811597685, -290.8272126874965693, -196.9803899876711739 ) ) ;
#37032=CARTESIAN_POINT ( 'NONE',  ( -60.33916665240547417, -283.8903411549292173, -199.7779612652877006 ) ) ;
#37035=CARTESIAN_POINT ( 'NONE',  ( -11.54911720562293631, -290.3877722157725998, -199.8803114367731837 ) ) ;
#37036=CARTESIAN_POINT ( 'NONE',  ( -64.60998207719204345, -279.0141852448809914, -338.9929373764626348 ) ) ;
#37037=CARTESIAN_POINT ( 'NONE',  ( -58.36297363748835920, -284.5229353502094796, -344.0784934699102564 ) ) ;
#37038=CARTESIAN_POINT ( 'NONE',  ( 37.30883395524732293, -273.4819731783036332, -258.5894353023925305 ) ) ;
#37039=CARTESIAN_POINT ( 'NONE',  ( -17.17187656040842469, -286.3197412667005892, -200.1500332567303815 ) ) ;
#37040=CARTESIAN_POINT ( 'NONE',  ( 1.195336417150171027, -277.9522902252868448, -333.1128814005253389 ) ) ;
#37041=CARTESIAN_POINT ( 'NONE',  ( -29.68638422648549735, -277.7557249646909554, -343.1720013271563516 ) ) ;
#37043=EDGE_CURVE ( 'NONE', #66639, #20110, #18660, .T. ) ;
#37044=CARTESIAN_POINT ( 'NONE',  ( -105.1853664718594104, -286.1318357377056145, -302.3335683525842228 ) ) ;
#37047=CARTESIAN_POINT ( 'NONE',  ( -88.60701418124442341, -295.5810413484387027, -327.8857968831457015 ) ) ;
#37048=CARTESIAN_POINT ( 'NONE',  ( -15.34337880032020962, -290.7460032282443194, -341.7448019072086254 ) ) ;
#37049=DIRECTION ( 'NONE',  ( 0.000000000000000000, 0.000000000000000000, -1.000000000000000000 ) ) ;
#37051=CARTESIAN_POINT ( 'NONE',  ( -2.659677404128715672, -276.9805209788415823, -198.2697987213421698 ) ) ;
#37052=CARTESIAN_POINT ( 'NONE',  ( -42.39589846619059443, -278.9101452985017886, -193.8369545496461797 ) ) ;
#37053=CARTESIAN_POINT ( 'NONE',  ( 3.778266276815157809, -292.9088607313422017, -334.5760871410036543 ) ) ;
#37054=CARTESIAN_POINT ( 'NONE',  ( -22.33740751207839281, -287.7677717395167178, -198.1590493296342856 ) ) ;
#37056=CARTESIAN_POINT ( 'NONE',  ( -110.2809383260595837, -280.1478595245853285, -282.9993998429006297 ) ) ;
#37057=CARTESIAN_POINT ( 'NONE',  ( 37.70801145274374022, -288.7964701229394677, -256.0032948246492310 ) ) ;
#37058=CARTESIAN_POINT ( 'NONE',  ( -77.16815995366074787, -285.5857159162177936, -333.9745020412080407 ) ) ;
#37059=CARTESIAN_POINT ( 'NONE',  ( -109.6069270068814632, -279.0565546539431239, -243.6226454669128998 ) ) ;
#37060=CARTESIAN_POINT ( 'NONE',  ( -72.41605985728138251, -295.6057489726476888, -204.4555097736812570 ) ) ;
#37061=CARTESIAN_POINT ( 'NONE',  ( 36.02963489785773987, -291.4018435801146438, -252.3067169072024001 ) ) ;
#37062=CARTESIAN_POINT ( 'NONE',  ( -75.00608125737090859, -279.3980205264095389, -203.2016480720518814 ) ) ;
#37063=CARTESIAN_POINT ( 'NONE',  ( -105.5234224581892590, -274.8020826622042136, -240.8689019982741115 ) ) ;
#37065=CARTESIAN_POINT ( 'NONE',  ( -95.95921662488163406, -286.4090924074130839, -317.1477375740089997 ) ) ;
#37066=CARTESIAN_POINT ( 'NONE',  ( -18.77557742772152594, -272.5277445104795220, -196.6232070001437080 ) ) ;
#37068=CARTESIAN_POINT ( 'NONE',  ( -89.51313367784943864, -278.8002414177943251, -219.1413082511308801 ) ) ;
#37069=CARTESIAN_POINT ( 'NONE',  ( 31.50518791976868016, -277.1920656444571591, -304.0694068053545607 ) ) ;
#37070=CARTESIAN_POINT ( 'NONE',  ( -93.20344372429528335, -298.6540565034932229, -222.4372358611114464 ) ) ;
#37071=CARTESIAN_POINT ( 'NONE',  ( -58.43364339371257898, -282.3769531223773583, -344.2266799187236188 ) ) ;
#37072=CARTESIAN_POINT ( 'NONE',  ( 35.00591514310363550, -289.5161752955698944, -286.0346310265603620 ) ) ;
#37073=CARTESIAN_POINT ( 'NONE',  ( 18.73489159201515974, -300.2623009399910075, -194.0402399066217640 ) ) ;
#37074=CARTESIAN_POINT ( 'NONE',  ( -68.03254280119637087, -298.8632833253699346, -200.1185621499464276 ) ) ;
#37075=CARTESIAN_POINT ( 'NONE',  ( -42.49107612656045774, -297.1174249618367753, -345.0170779197919160 ) ) ;
#37076=CARTESIAN_POINT ( 'NONE',  ( 19.88017639712701268, -280.2205166894802915, -318.6063603022816437 ) ) ;
#37077=CARTESIAN_POINT ( 'NONE',  ( -51.85716681453614285, -271.8857467313417828, -197.0883042514022918 ) ) ;
#37078=CARTESIAN_POINT ( 'NONE',  ( 24.04655775694280351, -288.5463040692736740, -225.2177661935517676 ) ) ;
#37079=CARTESIAN_POINT ( 'NONE',  ( -48.11995633477735623, -288.1126874506833815, -342.9248059595465747 ) ) ;
#37080=CARTESIAN_POINT ( 'NONE',  ( -108.9069067375272795, -267.5952716126691371, -307.0082179899138737 ) ) ;
#37082=CARTESIAN_POINT ( 'NONE',  ( -71.65823418849379323, -288.0714155168222419, -338.6325013365311634 ) ) ;
#37083=CARTESIAN_POINT ( 'NONE',  ( 34.03044012539324115, -287.4230921559598073, -285.8503994474906449 ) ) ;
#37085=CARTESIAN_POINT ( 'NONE',  ( -23.85383805456077155, -287.3001291021022894, -194.8116234015328416 ) ) ;
#37086=CARTESIAN_POINT ( 'NONE',  ( -35.11273941336074245, -277.3566764664938091, -343.3482347976537881 ) ) ;
#37087=CARTESIAN_POINT ( 'NONE',  ( -3.445535714056276788, -291.4094686568123507, -201.5531595875512210 ) ) ;
#37088=CARTESIAN_POINT ( 'NONE',  ( 30.62782783204197656, -281.7372433270249417, -234.2829683179864446 ) ) ;
#37089=CARTESIAN_POINT ( 'NONE',  ( -3.978391424313769242, -282.0042829910108821, -201.7202262214031521 ) ) ;
#37090=CARTESIAN_POINT ( 'NONE',  ( -50.08582698513463782, -283.5436691762438386, -346.3315869451657250 ) ) ;
#37091=CARTESIAN_POINT ( 'NONE',  ( 35.37298409981235636, -281.7902707737217156, -263.1450363258826997 ) ) ;
#37092=CARTESIAN_POINT ( 'NONE',  ( 84.90983274801601510, 83.18529645481817170, -302.4082324711995398 ) ) ;
#37093=CARTESIAN_POINT ( 'NONE',  ( -111.7927560011644914, -280.6559419418501307, -262.3084274197423156 ) ) ;
#37094=CARTESIAN_POINT ( 'NONE',  ( 188.3549636017863520, 271.3458732071474060, -139.1533289483813576 ) ) ;
#37095=CARTESIAN_POINT ( 'NONE',  ( -56.56367322532989306, -168.9367680551909814, -360.8783654570042927 ) ) ;
#37096=CARTESIAN_POINT ( 'NONE',  ( -65.86669663844585898, -272.8663103139484178, -202.9895638861965210 ) ) ;
#37097=CARTESIAN_POINT ( 'NONE',  ( 37.02471903805842857, -292.8120597285326312, -250.5830679493484183 ) ) ;
#37098=CARTESIAN_POINT ( 'NONE',  ( 189.7233545045971539, 267.9684856506630126, -137.6739583361996040 ) ) ;
#37099=CARTESIAN_POINT ( 'NONE',  ( -29.87027394958076698, -272.8296904090437351, -194.2199591836160266 ) ) ;
#37100=CARTESIAN_POINT ( 'NONE',  ( -26.37592589864985726, -287.3102865826921857, -343.3934915310548490 ) ) ;
#37101=CARTESIAN_POINT ( 'NONE',  ( -12.57417428062716169, -296.5872186386752105, -340.3969617874859637 ) ) ;
#37102=CARTESIAN_POINT ( 'NONE',  ( 34.77128114826058436, -289.0539340169237335, -284.6023332639597925 ) ) ;
#37104=CARTESIAN_POINT ( 'NONE',  ( -33.43478769535590800, -295.9453769504820571, -347.0394190793486473 ) ) ;
#37105=CARTESIAN_POINT ( 'NONE',  ( -37.28711696444914736, -286.5451654788275846, -197.2871505300908552 ) ) ;
#37106=CARTESIAN_POINT ( 'NONE',  ( -96.68808551110006988, -272.1274988696171704, -221.7659545690757739 ) ) ;
#37107=CARTESIAN_POINT ( 'NONE',  ( 39.06441415852493293, -294.2468602763872809, -261.7338714033780889 ) ) ;
#37108=CARTESIAN_POINT ( 'NONE',  ( 21.25949860412116621, -293.3715980453160341, -220.4869418272108135 ) ) ;
#37109=CARTESIAN_POINT ( 'NONE',  ( -95.11569292176378099, -291.3470766790228481, -225.7386375359353394 ) ) ;
#37110=ORIENTED_EDGE ( 'NONE', *, *, #49629, .T. ) ;
#37111=CARTESIAN_POINT ( 'NONE',  ( -30.00352153186533499, -276.0644967538614196, -195.1582900283677304 ) ) ;
#37112=CARTESIAN_POINT ( 'NONE',  ( 21.55545504677984425, -273.6848999524676174, -221.3801642117571475 ) ) ;
#37115=CARTESIAN_POINT ( 'NONE',  ( -111.7695086378747789, -277.8150088739178045, -289.9072141217940839 ) ) ;
#37116=CARTESIAN_POINT ( 'NONE',  ( 34.90869018961016934, -273.7549116749230507, -255.2553582066626063 ) ) ;
#37117=CARTESIAN_POINT ( 'NONE',  ( -9.547515864598405955, -274.8246755435575892, -339.2105763082400927 ) ) ;
#37118=CARTESIAN_POINT ( 'NONE',  ( -76.74189542565464706, -274.5906516487507361, -208.5399995537629820 ) ) ;
#37119=CARTESIAN_POINT ( 'NONE',  ( -81.22153907556885599, -274.3806759470620023, -211.6632869166898274 ) ) ;
#37120=CARTESIAN_POINT ( 'NONE',  ( -35.51649072041123389, -299.6747635556786236, -194.1606252097353718 ) ) ;
#37121=CARTESIAN_POINT ( 'NONE',  ( 36.60956285555379708, -273.3872414189284541, -255.8829444495767689 ) ) ;
#37122=CARTESIAN_POINT ( 'NONE',  ( -63.59786828688794458, -296.0549178954017862, -338.6386902729140616 ) ) ;
#37124=CARTESIAN_POINT ( 'NONE',  ( 34.64017021627132209, -292.3278390651728387, -285.7180687391007723 ) ) ;
#37126=CARTESIAN_POINT ( 'NONE',  ( -17.36782872132000932, -277.2934187614466737, -344.6616655181607030 ) ) ;
#37127=CARTESIAN_POINT ( 'NONE',  ( -31.34182623798868050, -274.2966847972199389, -197.5954511542159082 ) ) ;
#37129=CARTESIAN_POINT ( 'NONE',  ( -75.84396329312608032, -284.2345484348117566, -204.1875322436704607 ) ) ;
#37130=CARTESIAN_POINT ( 'NONE',  ( -111.3389064082464444, -298.7215197947444381, -257.1534728006878936 ) ) ;
#37132=CARTESIAN_POINT ( 'NONE',  ( -101.1271035063300019, -284.2397861864604351, -234.4240390724175711 ) ) ;
#37133=CARTESIAN_POINT ( 'NONE',  ( -106.2188952785525089, -276.4346918008217244, -297.4518174912482209 ) ) ;
#37134=CARTESIAN_POINT ( 'NONE',  ( -110.0771958099321779, -276.9806140440716717, -281.5379952495150064 ) ) ;
#37135=CARTESIAN_POINT ( 'NONE',  ( -31.02541847299138666, -284.9726307840362551, -345.1454264232606306 ) ) ;
#37136=CARTESIAN_POINT ( 'NONE',  ( 32.90083767457183939, -277.0380784229789128, -291.6912475501101198 ) ) ;
#37138=CARTESIAN_POINT ( 'NONE',  ( 37.11953329148045100, -274.1573449175235169, -286.6073447017477065 ) ) ;
#37139=CARTESIAN_POINT ( 'NONE',  ( -95.41760529303932969, -281.2091043533106927, -222.6208934255556358 ) ) ;
#37141=CARTESIAN_POINT ( 'NONE',  ( -10.52827084031595639, -288.3192551652211364, -199.6629480257257114 ) ) ;
#37143=CARTESIAN_POINT ( 'NONE',  ( 32.23614578605712921, -291.9184178325068046, -298.4963633471092521 ) ) ;
#37144=CARTESIAN_POINT ( 'NONE',  ( 82.17437182012335484, -297.5505941057896280, -195.5323370396037035 ) ) ;
#37145=CARTESIAN_POINT ( 'NONE',  ( -55.37646185865559545, -296.6099646319331100, -199.1616506149183010 ) ) ;
#37146=CARTESIAN_POINT ( 'NONE',  ( -109.5574381313751644, -288.4686289342589589, -287.5585790842105780 ) ) ;
#37147=CARTESIAN_POINT ( 'NONE',  ( 189.0118003482855613, 275.4351431090623237, -122.7278359107281887 ) ) ;
#37148=CARTESIAN_POINT ( 'NONE',  ( -37.81013033203306861, -296.0461271000310148, -195.3625764867553016 ) ) ;
#37149=CARTESIAN_POINT ( 'NONE',  ( -41.74011743944212327, -287.5864703687000201, -346.5540194227464212 ) ) ;
#37150=CARTESIAN_POINT ( 'NONE',  ( -8.159353768194760548, -284.2635759339248125, -338.1463013005608218 ) ) ;
#37151=CARTESIAN_POINT ( 'NONE',  ( -95.03233181523984285, -283.4689498841880777, -220.8275482326354506 ) ) ;
#37152=CARTESIAN_POINT ( 'NONE',  ( -45.68841944365056662, -284.5851508454682630, -343.5268660307907567 ) ) ;
#37153=CARTESIAN_POINT ( 'NONE',  ( -58.98617070704653997, -284.1421791984462857, -340.3008443430176158 ) ) ;
#37154=CARTESIAN_POINT ( 'NONE',  ( -71.14553320370634992, -291.4760290429610450, -337.7087807191740012 ) ) ;
#37155=CARTESIAN_POINT ( 'NONE',  ( -88.02564103446042054, -273.6993168240351793, -212.3516357369291825 ) ) ;
#37156=CARTESIAN_POINT ( 'NONE',  ( 17.58100758195860536, -286.3542267474915661, -322.2534139018941346 ) ) ;
#37157=CARTESIAN_POINT ( 'NONE',  ( 13.96447640051007610, -274.7484070352196568, -212.8731763715531144 ) ) ;
#37158=CARTESIAN_POINT ( 'NONE',  ( 35.24135088202188371, -295.3066135317819203, -252.8839762770671484 ) ) ;
#37160=CARTESIAN_POINT ( 'NONE',  ( 10.64812456238590066, -290.9090924074130839, -330.4860931364851808 ) ) ;
#37161=CARTESIAN_POINT ( 'NONE',  ( -59.11007243505797959, -282.0245136325808630, -340.6099320266833388 ) ) ;
#37162=CARTESIAN_POINT ( 'NONE',  ( -83.75484944032145052, -275.6869242708368120, -329.5529688687923908 ) ) ;
#37163=CARTESIAN_POINT ( 'NONE',  ( -98.99531427405814554, -271.6352340948325832, -225.3119947928427109 ) ) ;
#37164=CARTESIAN_POINT ( 'NONE',  ( 26.85230179668491601, -275.3787197170688614, -305.4386597724418380 ) ) ;
#37165=CARTESIAN_POINT ( 'NONE',  ( 21.53618899909647055, -294.4557530579195941, -226.0429284211115259 ) ) ;
#37166=CARTESIAN_POINT ( 'NONE',  ( 0.01880844349002916416, -293.5039402878927035, -207.3722233468175773 ) ) ;
#37167=CARTESIAN_POINT ( 'NONE',  ( -107.1217038909655912, -285.9866456125935770, -295.1859555809152766 ) ) ;
#37168=EDGE_CURVE ( 'NONE', #47196, #64642, #50429, .T. ) ;
#37169=CARTESIAN_POINT ( 'NONE',  ( 36.53159358878502871, -295.2237751869107569, -289.8891176156973870 ) ) ;
#37170=CARTESIAN_POINT ( 'NONE',  ( 24.40646849695092513, -294.2637080330470098, -225.1896452906121624 ) ) ;
#37171=CARTESIAN_POINT ( 'NONE',  ( -69.72597773767806473, -295.3242280397142281, -335.7848030533413635 ) ) ;
#37172=CARTESIAN_POINT ( 'NONE',  ( -72.07701453124620627, -291.5116069881614749, -336.8471122894359837 ) ) ;
#37173=CARTESIAN_POINT ( 'NONE',  ( -52.91553849778298257, -283.4129980048540460, -345.8242004598414496 ) ) ;
#37174=CARTESIAN_POINT ( 'NONE',  ( -20.87629721956141893, -296.3365913390894661, -194.8064469063934894 ) ) ;
#37175=CARTESIAN_POINT ( 'NONE',  ( -65.87538817740572483, -285.5223501403916657, -198.8289333778589025 ) ) ;
#37176=CARTESIAN_POINT ( 'NONE',  ( -79.54156228122062089, -279.6047886331531345, -331.9952902659023266 ) ) ;
#37178=CARTESIAN_POINT ( 'NONE',  ( -57.48872647716817852, -284.5812856528338557, -199.7304081365564628 ) ) ;
#37179=CARTESIAN_POINT ( 'NONE',  ( 25.74824362719364146, -286.0993400141191501, -311.0112308093402476 ) ) ;
#37180=CARTESIAN_POINT ( 'NONE',  ( -56.22551449035876203, -277.9511249168207883, -196.9332559652179668 ) ) ;
#37182=CARTESIAN_POINT ( 'NONE',  ( -108.4866588822361280, -283.8400249096803236, -287.0405797903704297 ) ) ;
#37183=CARTESIAN_POINT ( 'NONE',  ( 37.48101548385013615, -282.9643855393206309, -286.8403346246170145 ) ) ;
#37184=CARTESIAN_POINT ( 'NONE',  ( -29.01465186027991905, -288.0079456625308580, -346.7262120174191296 ) ) ;
#37185=CARTESIAN_POINT ( 'NONE',  ( -82.06016339930624781, -279.2508283923674526, -332.0595738483911532 ) ) ;
#37186=CARTESIAN_POINT ( 'NONE',  ( -35.70515885984242743, -278.3472253223114876, -346.8635030127408072 ) ) ;
#37187=CARTESIAN_POINT ( 'NONE',  ( -72.12783937481628982, -279.4117044711398421, -206.1822700587617021 ) ) ;
#37188=CARTESIAN_POINT ( 'NONE',  ( -46.40289275953759329, -275.9164964099653048, -196.2683275814586068 ) ) ;
#37189=CARTESIAN_POINT ( 'NONE',  ( 11.11878729026226686, -292.7017228325184419, -210.4545615941174219 ) ) ;
#37190=CARTESIAN_POINT ( 'NONE',  ( 19.05196499571339785, -286.2545813980258913, -319.3424753718862803 ) ) ;
#37192=CARTESIAN_POINT ( 'NONE',  ( -107.6370626030929571, -292.5302789497656022, -240.9501943634475651 ) ) ;
#37193=CARTESIAN_POINT ( 'NONE',  ( 21.56669368202042847, -293.0817289457330617, -313.9962782670322099 ) ) ;
#37194=CARTESIAN_POINT ( 'NONE',  ( -28.89774648281880687, -294.6090157395627784, -342.9434300135208673 ) ) ;
#37195=CARTESIAN_POINT ( 'NONE',  ( -113.0526920475670352, -291.4783708322835309, -282.5815194711419167 ) ) ;
#37196=CARTESIAN_POINT ( 'NONE',  ( 33.05984951545999451, -282.4633875713348630, -290.0465053594404594 ) ) ;
#37197=CARTESIAN_POINT ( 'NONE',  ( -46.08094623810074353, -296.8641019593885062, -194.1697924476801518 ) ) ;
#37198=CARTESIAN_POINT ( 'NONE',  ( 37.04791602180043952, -288.4477338975623866, -289.8418211521286594 ) ) ;
#37199=CARTESIAN_POINT ( 'NONE',  ( 12.84458278802912190, -280.5005193778989110, -327.1904458860697673 ) ) ;
#37200=CARTESIAN_POINT ( 'NONE',  ( 35.05403498052020694, -288.2177055046319651, -296.6811252165226165 ) ) ;
#37201=CARTESIAN_POINT ( 'NONE',  ( -49.42920682756628281, -286.2272189558863715, -198.2958577122393820 ) ) ;
#37202=CARTESIAN_POINT ( 'NONE',  ( 179.6752721478330557, 254.2973581424797374, -166.6431896918319637 ) ) ;
#37203=CARTESIAN_POINT ( 'NONE',  ( -64.79168948216373281, -181.8610138526347839, -360.2174547310475532 ) ) ;
#37204=CARTESIAN_POINT ( 'NONE',  ( -76.76410942417290073, -208.0616896646858152, -353.4147769976461291 ) ) ;
#37205=CARTESIAN_POINT ( 'NONE',  ( -110.0657075408640821, -277.6382604475187463, -278.7983081019125393 ) ) ;
#37206=CARTESIAN_POINT ( 'NONE',  ( -92.97013546518614646, -276.7955974803167578, -318.1073561200034874 ) ) ;
#37207=CARTESIAN_POINT ( 'NONE',  ( 30.72698958417520387, -298.3906325157475976, -193.4281377556751522 ) ) ;
#37208=CARTESIAN_POINT ( 'NONE',  ( 200.4462836145382312, 285.9195334705995606, -96.58237528659300608 ) ) ;
#37209=CARTESIAN_POINT ( 'NONE',  ( -22.66146481047934813, -278.8110956830652185, -195.3199634834428196 ) ) ;
#37210=CARTESIAN_POINT ( 'NONE',  ( 22.38921990735957479, -295.9489660591522693, -317.3521110250798642 ) ) ;
#37211=CARTESIAN_POINT ( 'NONE',  ( -4.811308010211996056, -292.9848514098938494, -204.9272918964365147 ) ) ;
#37212=CARTESIAN_POINT ( 'NONE',  ( -97.63572512416159555, -274.1307999741873118, -222.8484800435509499 ) ) ;
#37213=CARTESIAN_POINT ( 'NONE',  ( 6.122885099020168198, -287.1335185242441526, -329.6872779768310693 ) ) ;
#37214=CARTESIAN_POINT ( 'NONE',  ( 30.71440275779965035, -299.3751842690778062, -193.4171149168752493 ) ) ;
#37215=CARTESIAN_POINT ( 'NONE',  ( -81.94579477330741213, -297.5917719608419816, -212.5088625246573315 ) ) ;
#37218=CARTESIAN_POINT ( 'NONE',  ( -53.47727111639837005, -281.7670297583512706, -196.4905116048815614 ) ) ;
#37219=CARTESIAN_POINT ( 'NONE',  ( -110.6607936354956792, -279.6640070631573280, -267.9115927433266506 ) ) ;
#37220=CARTESIAN_POINT ( 'NONE',  ( -109.5932499090205710, -280.6141581524346407, -246.6633948029254668 ) ) ;
#37221=CARTESIAN_POINT ( 'NONE',  ( 0.9894731810292046736, -273.0536950562868128, -207.4212347213027101 ) ) ;
#37226=CARTESIAN_POINT ( 'NONE',  ( -64.81808472547032807, -279.8497032214888236, -202.7294072695395926 ) ) ;
#37227=CARTESIAN_POINT ( 'NONE',  ( 32.87635832453768359, -276.7540506009354999, -301.5634109616956948 ) ) ;
#37228=CARTESIAN_POINT ( 'NONE',  ( 35.95664103302951276, -277.7570510616286583, -286.3068623283666057 ) ) ;
#37229=CARTESIAN_POINT ( 'NONE',  ( -62.23134649491931469, -275.9442275230288715, -342.6604208264586191 ) ) ;
#37232=CARTESIAN_POINT ( 'NONE',  ( -13.90895442258618431, -284.7294743734213398, -341.9803418662686454 ) ) ;
#37233=CARTESIAN_POINT ( 'NONE',  ( -81.81912626926953180, -290.6259927298177104, -212.2077736812288435 ) ) ;
#37234=CARTESIAN_POINT ( 'NONE',  ( 38.45779427508252724, -286.7375759682649914, -257.3317933329411176 ) ) ;
#37235=CARTESIAN_POINT ( 'NONE',  ( -65.72474233370687102, -281.6683844946635418, -338.7296945338605383 ) ) ;
#37236=CARTESIAN_POINT ( 'NONE',  ( 8.144035905089078042, -280.9911625579424026, -328.2744583910110237 ) ) ;
#37237=CARTESIAN_POINT ( 'NONE',  ( 35.11753903505927354, -285.4106169121541825, -253.2480271490028940 ) ) ;
#37238=CARTESIAN_POINT ( 'NONE',  ( 31.43704377151221863, -282.4155690147152313, -244.5908916414939824 ) ) ;
#37239=CARTESIAN_POINT ( 'NONE',  ( -112.3417001280813565, -270.5523135751784594, -270.3357089863371812 ) ) ;
#37240=CARTESIAN_POINT ( 'NONE',  ( -70.14439826573801895, -281.8769492942743113, -339.1535044043376388 ) ) ;
#37241=CARTESIAN_POINT ( 'NONE',  ( -22.46859069622999527, -296.8618801463102272, -343.8716020072762944 ) ) ;
#37242=CARTESIAN_POINT ( 'NONE',  ( -74.63590070761051720, -280.4843582892498262, -207.2746477157267577 ) ) ;
#37243=CARTESIAN_POINT ( 'NONE',  ( -94.44099627240861139, -287.2286414266218912, -221.3984778033835710 ) ) ;
#37245=CARTESIAN_POINT ( 'NONE',  ( -78.82466731291643214, -293.4184390265403977, -207.1441659699051741 ) ) ;
#37246=CARTESIAN_POINT ( 'NONE',  ( 8.791087937605919223, -274.4199449409945260, -329.5607401776369443 ) ) ;
#37247=CARTESIAN_POINT ( 'NONE',  ( 10.12015998139964523, -287.6141237037815017, -330.8566964078613069 ) ) ;
#37248=CARTESIAN_POINT ( 'NONE',  ( 35.70242817470591490, -291.8145452261563833, -259.8256666000236805 ) ) ;
#37249=CARTESIAN_POINT ( 'NONE',  ( -98.06567382502505836, -276.6649003716942730, -311.7596988370123086 ) ) ;
#37250=CARTESIAN_POINT ( 'NONE',  ( -109.6753463270026003, -294.9083027293222585, -253.6665346802094518 ) ) ;
#37251=CARTESIAN_POINT ( 'NONE',  ( -110.8615624681319645, -291.8921702570154366, -268.4656389857661907 ) ) ;
#37253=CARTESIAN_POINT ( 'NONE',  ( -41.92345788835077514, -293.5886472342795059, -346.5820305606991951 ) ) ;
#37254=CARTESIAN_POINT ( 'NONE',  ( 33.79502637761630268, -288.8954811245253609, -250.7140683692962284 ) ) ;
#37255=CARTESIAN_POINT ( 'NONE',  ( -112.6586249066970140, -288.9244592299990586, -259.9102210491147957 ) ) ;
#37256=CARTESIAN_POINT ( 'NONE',  ( 34.27870761690637380, -289.1987015317446890, -287.2694624750785124 ) ) ;
#37258=CARTESIAN_POINT ( 'NONE',  ( -82.63825224533155733, -290.4924902514837868, -327.8139168065159765 ) ) ;
#37260=CARTESIAN_POINT ( 'NONE',  ( -80.30515343051358457, -290.8247594925233557, -333.8456154741436990 ) ) ;
#37261=CARTESIAN_POINT ( 'NONE',  ( -4.354366754540068385, -278.5048357423264633, -202.5955776277986615 ) ) ;
#37262=CARTESIAN_POINT ( 'NONE',  ( -104.7771072349043067, -279.3664035069019178, -233.2368649963776477 ) ) ;
#37263=CARTESIAN_POINT ( 'NONE',  ( 8.537341559538260682, -280.3278088705010873, -208.4817666927683604 ) ) ;
#37264=CARTESIAN_POINT ( 'NONE',  ( 35.33271381935216482, -285.3133092422007167, -251.7773406110986798 ) ) ;
#37266=CARTESIAN_POINT ( 'NONE',  ( 12.14659068537289599, -278.8889627864730301, -215.0278138133120649 ) ) ;
#37267=CARTESIAN_POINT ( 'NONE',  ( -6.306978966449482193, -280.6442960714742867, -338.6388356855028974 ) ) ;
#37268=CARTESIAN_POINT ( 'NONE',  ( -88.01846039707731961, -229.9137307660017484, -344.5856827696274536 ) ) ;
#37269=CARTESIAN_POINT ( 'NONE',  ( -111.8120368226499295, -276.8220449022496155, -287.0007306086178573 ) ) ;
#37270=CARTESIAN_POINT ( 'NONE',  ( -111.4190244139907122, -283.7243002278159452, -250.3111566686916376 ) ) ;
#37271=CARTESIAN_POINT ( 'NONE',  ( -35.82142624576487577, -299.0128965477977090, -197.1255714116523734 ) ) ;
#37272=CARTESIAN_POINT ( 'NONE',  ( -80.92927823114250430, -274.8987345943192508, -207.5376944864815982 ) ) ;
#37273=CARTESIAN_POINT ( 'NONE',  ( 35.39967989315321262, -275.1273696347490727, -263.4229568557001926 ) ) ;
#37274=CARTESIAN_POINT ( 'NONE',  ( -28.63930020621857153, -296.9420813785833388, -344.9069457492344100 ) ) ;
#37275=CARTESIAN_POINT ( 'NONE',  ( 16.68746894093080968, -288.4760545915963235, -325.2973537541544715 ) ) ;
#37276=CARTESIAN_POINT ( 'NONE',  ( 26.64518807274798462, -279.0946793915359763, -230.0760469442941201 ) ) ;
#37277=CARTESIAN_POINT ( 'NONE',  ( -67.01348336552244689, -291.5071411942748227, -199.3077205688790627 ) ) ;
#37278=CARTESIAN_POINT ( 'NONE',  ( -103.0618413403168177, -289.1744323941791777, -302.6763076990845320 ) ) ;
#37279=CARTESIAN_POINT ( 'NONE',  ( 36.62938245601388587, -291.7119545675024597, -282.8193912004442154 ) ) ;
#37282=CARTESIAN_POINT ( 'NONE',  ( -108.7241931824519554, -289.8538284535074467, -285.9926154946443830 ) ) ;
#37284=CARTESIAN_POINT ( 'NONE',  ( -36.57984325276299842, -287.0027419501200256, -193.5871929265269102 ) ) ;
#37285=CARTESIAN_POINT ( 'NONE',  ( -53.28691492658256834, -297.7662352645559167, -340.3683826091709079 ) ) ;
#37286=CARTESIAN_POINT ( 'NONE',  ( -27.78903667325146287, -293.9925540688091701, -346.5822642311194954 ) ) ;
#37287=CARTESIAN_POINT ( 'NONE',  ( -0.5974777997168068122, -283.8896200043104727, -337.4815542766774570 ) ) ;
#37288=CARTESIAN_POINT ( 'NONE',  ( -105.2147187587827091, -284.0243312394444501, -297.3735001381943448 ) ) ;
#37289=CARTESIAN_POINT ( 'NONE',  ( 20.23144391921339036, -276.2266426169885563, -224.6619271695542466 ) ) ;
#37290=CARTESIAN_POINT ( 'NONE',  ( 35.67126341593337457, -291.7733089069558901, -285.9450239843537815 ) ) ;
#37292=CARTESIAN_POINT ( 'NONE',  ( -69.65200492506903629, -272.4118915382899786, -204.4583508926859565 ) ) ;
#37294=CARTESIAN_POINT ( 'NONE',  ( -108.4555765497910471, -262.4588243622614527, -317.8183916042563055 ) ) ;
#37295=CARTESIAN_POINT ( 'NONE',  ( 38.33568392662063218, -293.3960930538071352, -284.5276334989173961 ) ) ;
#37296=CARTESIAN_POINT ( 'NONE',  ( 30.10454924828650292, -289.0551557443410502, -238.8600443507633031 ) ) ;
#37297=CARTESIAN_POINT ( 'NONE',  ( -88.38938719997088356, -296.8271921599790062, -327.6654055070242180 ) ) ;
#37298=CARTESIAN_POINT ( 'NONE',  ( -2.144580861112217463, -287.1822253493394896, -206.2336185821078800 ) ) ;
#37299=CARTESIAN_POINT ( 'NONE',  ( -111.9493516628153600, -277.3835340378610113, -288.4860338994133713 ) ) ;
#37300=CARTESIAN_POINT ( 'NONE',  ( 19.45999875845602745, -294.9099003179920828, -322.2738091659118140 ) ) ;
#37301=CARTESIAN_POINT ( 'NONE',  ( 19.62821790832263247, -286.3787296932925415, -320.3279667410840830 ) ) ;
#37302=CARTESIAN_POINT ( 'NONE',  ( -33.43166539612342802, -295.3375043451268311, -347.2537233179010059 ) ) ;
#37303=CARTESIAN_POINT ( 'NONE',  ( -60.26963068164201331, -292.0799649252532504, -200.9798745687502048 ) ) ;
#37306=CARTESIAN_POINT ( 'NONE',  ( 153.8785610233898353, 204.4371874965355005, -214.4256267419547157 ) ) ;
#37307=CARTESIAN_POINT ( 'NONE',  ( -15.62943896399615262, -287.8481154429661615, -197.1537483369301640 ) ) ;
#37308=CARTESIAN_POINT ( 'NONE',  ( 25.22466315766302358, -290.4094976428775112, -220.5068182859052968 ) ) ;
#37309=EDGE_LOOP ( 'NONE', ( #53841, #31143, #16046, #17128 ) ) ;
#37310=CARTESIAN_POINT ( 'NONE',  ( -45.25462026394541937, -279.3031421062002551, -193.8183392458116145 ) ) ;
#37311=CARTESIAN_POINT ( 'NONE',  ( 18.41213393662922826, -282.8556198275064162, -220.4458055518025503 ) ) ;
#37312=CARTESIAN_POINT ( 'NONE',  ( 204.7385621006099541, 293.0224724744894615, -54.00000000000019185 ) ) ;
#37313=CARTESIAN_POINT ( 'NONE',  ( -89.47089566606882727, -283.9099361480904804, -214.4218883608680244 ) ) ;
#37314=CARTESIAN_POINT ( 'NONE',  ( -42.79331104629897453, -287.2011782544228140, -344.6528317607025542 ) ) ;
#37315=CARTESIAN_POINT ( 'NONE',  ( -0.6644879575998082766, -276.3944040201157009, -204.0509106616867712 ) ) ;
#37316=CARTESIAN_POINT ( 'NONE',  ( -109.1073012028064113, -297.2259518018898916, -256.5945685722813323 ) ) ;
#37317=CARTESIAN_POINT ( 'NONE',  ( 14.65341603429722284, -292.9863700605037593, -322.3725373520155131 ) ) ;
#37318=CARTESIAN_POINT ( 'NONE',  ( -113.6170953225393561, -279.3309410343756554, -260.1895831718448449 ) ) ;
#37319=CARTESIAN_POINT ( 'NONE',  ( 32.51638969446961624, -275.8331972023412391, -291.5904667548300608 ) ) ;
#37320=CARTESIAN_POINT ( 'NONE',  ( -68.73017754652568101, -274.7288321063439867, -200.3735272335182174 ) ) ;
#37321=CARTESIAN_POINT ( 'NONE',  ( -23.01020350233489609, -275.7934125632637006, -345.7549851419325364 ) ) ;
#37323=CARTESIAN_POINT ( 'NONE',  ( 37.70720199943995965, -273.5442517067217523, -269.7586664074857481 ) ) ;
#37324=CARTESIAN_POINT ( 'NONE',  ( -112.3141080162607324, -298.1642372451777874, -255.5375871175444331 ) ) ;
#37325=CARTESIAN_POINT ( 'NONE',  ( -112.3417001280813849, -275.0519495502701943, -270.3929463913696054 ) ) ;
#37327=CARTESIAN_POINT ( 'NONE',  ( -54.84340659790353101, -286.9016483771832782, -199.1192969965702559 ) ) ;
#37328=CARTESIAN_POINT ( 'NONE',  ( -85.44336532270544637, -285.4669562479273281, -329.1846151312274742 ) ) ;
#37329=CARTESIAN_POINT ( 'NONE',  ( -65.12428514459263340, -285.0280038265851772, -202.6905196007719212 ) ) ;
#37330=CARTESIAN_POINT ( 'NONE',  ( -93.34689749296420302, -276.2752246297795296, -318.4221030415608311 ) ) ;
#37331=CARTESIAN_POINT ( 'NONE',  ( -69.52356149078943304, -285.3407113747234121, -337.2720372971938900 ) ) ;
#37332=CARTESIAN_POINT ( 'NONE',  ( -110.8488725689581429, -277.1004294037684872, -265.1262969920673527 ) ) ;
#37333=EDGE_CURVE ( 'NONE', #78639, #9799, #560, .T. ) ;
#37334=CARTESIAN_POINT ( 'NONE',  ( -29.66745107731571096, -278.0325191603734538, -343.3185633340101504 ) ) ;
#37335=EDGE_CURVE ( 'NONE', #57853, #60383, #89729, .T. ) ;
#37337=CARTESIAN_POINT ( 'NONE',  ( -110.4034719488357297, -273.0803523630808627, -267.6412165631991797 ) ) ;
#37338=CARTESIAN_POINT ( 'NONE',  ( 19.03472298386827433, -281.6422731844011764, -218.1513704480079241 ) ) ;
#37339=CARTESIAN_POINT ( 'NONE',  ( -5.475280587860151371, -283.1364005535865545, -340.3900991914817951 ) ) ;
#37343=CARTESIAN_POINT ( 'NONE',  ( 22.00925704606999034, -288.7718418219653245, -223.2472496350641791 ) ) ;
#37344=CARTESIAN_POINT ( 'NONE',  ( -111.4485672590603826, -288.9969268384077736, -289.4259508522750366 ) ) ;
#37345=CARTESIAN_POINT ( 'NONE',  ( -75.28566730507230886, -296.7298162703662001, -207.7495515911309383 ) ) ;
#37346=CARTESIAN_POINT ( 'NONE',  ( -69.57285839711249764, -290.9875572401598447, -200.5294255433047113 ) ) ;
#37347=CARTESIAN_POINT ( 'NONE',  ( 34.06515417399135970, -285.7932701412069605, -252.0956060185467038 ) ) ;
#37348=CARTESIAN_POINT ( 'NONE',  ( -76.19512105307381944, -288.1573354591596399, -332.8574106658682012 ) ) ;
#37349=CARTESIAN_POINT ( 'NONE',  ( -35.94119580413624249, -287.2751839588753455, -196.9774066180032719 ) ) ;
#37350=CARTESIAN_POINT ( 'NONE',  ( -109.8992335756570498, -276.3074393677642320, -289.3959833164004749 ) ) ;
#37351=CARTESIAN_POINT ( 'NONE',  ( -8.965592794820878453, -290.6812121732749574, -339.7997750843401832 ) ) ;
#37352=CARTESIAN_POINT ( 'NONE',  ( -73.56668085324497497, -287.5314850686552290, -336.2376344362913301 ) ) ;
#37353=CARTESIAN_POINT ( 'NONE',  ( -98.30956833429530661, -286.0548376537249737, -229.7861565585783978 ) ) ;
#37354=CARTESIAN_POINT ( 'NONE',  ( -100.1660193917986987, -293.1090998540954047, -228.9986340924901072 ) ) ;
#37357=CARTESIAN_POINT ( 'NONE',  ( -96.53699812076511932, -275.1692720078602292, -223.7314760895574466 ) ) ;
#37358=CARTESIAN_POINT ( 'NONE',  ( -43.75507891956904416, -279.1663383484598171, -197.4309382420261159 ) ) ;
#37359=CARTESIAN_POINT ( 'NONE',  ( 34.87863396652471693, -279.8122422810128000, -290.5904035344075282 ) ) ;
#37360=CARTESIAN_POINT ( 'NONE',  ( 11.08859352418373412, -293.5985985249304804, -330.0842288860447979 ) ) ;
#37361=CARTESIAN_POINT ( 'NONE',  ( -64.92591828202790794, -271.9267068637113312, -201.6664154785643746 ) ) ;
#37362=CARTESIAN_POINT ( 'NONE',  ( 17.57733476761621461, -274.3391491081213189, -320.6316280927646858 ) ) ;
#37363=CARTESIAN_POINT ( 'NONE',  ( -50.05558065664418876, -299.2016873674821227, -197.9760316823304720 ) ) ;
#37365=CARTESIAN_POINT ( 'NONE',  ( -113.2957492518303155, -294.8376403577980795, -266.7606426456421786 ) ) ;
#37366=CARTESIAN_POINT ( 'NONE',  ( 36.29771464335428988, -294.9824560454705988, -270.7450278594627093 ) ) ;
#37367=CARTESIAN_POINT ( 'NONE',  ( -94.89414429562873465, -296.7194265151134687, -315.5309961967191725 ) ) ;
#37369=CARTESIAN_POINT ( 'NONE',  ( -43.50602473436414641, -283.9948892174213597, -195.2063478201638986 ) ) ;
#37370=CARTESIAN_POINT ( 'NONE',  ( -97.18337698819165382, -295.9691845535620018, -312.1698935036170610 ) ) ;
#37371=CARTESIAN_POINT ( 'NONE',  ( -71.73874023561099023, -283.4941621538452523, -339.2512016800052379 ) ) ;
#37372=CARTESIAN_POINT ( 'NONE',  ( 14.77826650365005179, -284.2448253073169440, -325.0678202639791721 ) ) ;
#37373=CARTESIAN_POINT ( 'NONE',  ( -33.72407509847515428, -285.7632304212094141, -193.4673140662763728 ) ) ;
#37374=CARTESIAN_POINT ( 'NONE',  ( 33.54571662535364140, -291.2393223265788720, -246.2204340254771466 ) ) ;
#37375=CARTESIAN_POINT ( 'NONE',  ( -114.1306607305792085, -277.8494598791134536, -274.4560313994116427 ) ) ;
#37376=CARTESIAN_POINT ( 'NONE',  ( 39.58706461736020543, -273.0523547857347353, -270.3937649182068981 ) ) ;
#37378=CARTESIAN_POINT ( 'NONE',  ( 13.42522107200286463, -285.5764883299042367, -217.2829634672676207 ) ) ;
#37379=CARTESIAN_POINT ( 'NONE',  ( -113.8054590362175134, -289.3902066666066162, -276.9134418955106867 ) ) ;
#37381=CARTESIAN_POINT ( 'NONE',  ( -101.9243865285431241, -298.6350917238896159, -234.6467366958367506 ) ) ;
#37382=CARTESIAN_POINT ( 'NONE',  ( -92.89304552555748273, -279.2547832978563065, -322.9027667087220266 ) ) ;
#37383=CARTESIAN_POINT ( 'NONE',  ( -30.76026802195017851, -292.9894435751852484, -345.4283648619525593 ) ) ;
#37384=CARTESIAN_POINT ( 'NONE',  ( 26.87162744191877906, -281.6931065999290240, -305.1279994803028899 ) ) ;
#37385=CARTESIAN_POINT ( 'NONE',  ( 37.46051242382480950, -293.9479373214531961, -288.6818090625475293 ) ) ;
#37386=CARTESIAN_POINT ( 'NONE',  ( -7.881574408821461653, -284.5148489674409689, -200.7252337286944339 ) ) ;
#37387=CARTESIAN_POINT ( 'NONE',  ( -100.2285193883173235, -281.1044126408368697, -229.3984215881124840 ) ) ;
#37388=CARTESIAN_POINT ( 'NONE',  ( 1.685113069783463979, -293.5753743016081216, -332.3914583416751043 ) ) ;
#37389=CARTESIAN_POINT ( 'NONE',  ( -35.85140150718095953, -296.0706510178139297, -195.3616173567541807 ) ) ;
#37392=CARTESIAN_POINT ( 'NONE',  ( 35.25562079966431384, -283.7567442868192984, -287.7786304767633396 ) ) ;
#37393=CARTESIAN_POINT ( 'NONE',  ( -103.9953280096532779, -295.6556189317900589, -300.4060806146274558 ) ) ;
#37395=CARTESIAN_POINT ( 'NONE',  ( -112.3381139276884824, -270.1608578419545097, -261.8788190812425114 ) ) ;
#37396=CARTESIAN_POINT ( 'NONE',  ( -52.50373260795684871, -273.0600028258471639, -194.9790315404535477 ) ) ;
#37397=CARTESIAN_POINT ( 'NONE',  ( -101.6441519101626483, -289.9129493538187603, -305.0254202082359143 ) ) ;
#37398=CARTESIAN_POINT ( 'NONE',  ( -109.5706370151317088, -280.2641284949510805, -255.6795837693958049 ) ) ;
#37399=CARTESIAN_POINT ( 'NONE',  ( 3.354289148334625548, -276.2089456547820419, -208.7348288689008200 ) ) ;
#37400=CARTESIAN_POINT ( 'NONE',  ( -35.89374908788306584, -284.6344323884651430, -346.5603429344531037 ) ) ;
#37401=CARTESIAN_POINT ( 'NONE',  ( -41.05601463738571510, -278.7992868972816041, -197.0580868500661893 ) ) ;
#37402=CARTESIAN_POINT ( 'NONE',  ( -62.43563910140775874, -279.3786325067005123, -341.0937236069890446 ) ) ;
#37404=CARTESIAN_POINT ( 'NONE',  ( -66.22525101921424096, -273.5176931674315028, -198.9694971214037764 ) ) ;
#37405=CARTESIAN_POINT ( 'NONE',  ( -96.26901032218887622, -293.1002669520462405, -224.8761060050186984 ) ) ;
#37407=DIRECTION ( 'NONE',  ( 1.000000000000000000, 0.000000000000000000, 0.000000000000000000 ) ) ;
#37408=CARTESIAN_POINT ( 'NONE',  ( 38.26770867222952432, -291.7630473726748050, -275.9716602547186426 ) ) ;
#37409=CARTESIAN_POINT ( 'NONE',  ( -54.21967317918562657, -273.3371222145809725, -199.2757997576158289 ) ) ;
#37411=CARTESIAN_POINT ( 'NONE',  ( -8.788781319167595640, -293.9391410176762633, -199.5978607045482534 ) ) ;
#37412=CARTESIAN_POINT ( 'NONE',  ( -85.28047601435908120, -280.1948066931273047, -330.5268031993605859 ) ) ;
#37413=CARTESIAN_POINT ( 'NONE',  ( -30.74682907686137057, -293.3387003487656557, -193.9901124214263461 ) ) ;
#37414=CARTESIAN_POINT ( 'NONE',  ( 18.23554217258606513, -288.8521129944070935, -220.2301350138416183 ) ) ;
#37415=CARTESIAN_POINT ( 'NONE',  ( 36.65831020759688386, -273.4075654051913489, -259.1379700485984472 ) ) ;
#37416=CARTESIAN_POINT ( 'NONE',  ( 33.47549543653630622, -277.7707624468934000, -293.3010179413162746 ) ) ;
#37417=CARTESIAN_POINT ( 'NONE',  ( 35.47108514671395341, -291.8330373702094676, -285.9015887351851575 ) ) ;
#37418=CARTESIAN_POINT ( 'NONE',  ( -96.74347011726838730, -281.0521018647543201, -223.3320290363749052 ) ) ;
#37420=CARTESIAN_POINT ( 'NONE',  ( -88.91222810340087790, -283.4677924453893638, -322.1289812723898649 ) ) ;
#37421=CARTESIAN_POINT ( 'NONE',  ( 14.94051194281458272, -281.8481122527446701, -214.1809348605969205 ) ) ;
#37422=CARTESIAN_POINT ( 'NONE',  ( -83.65540756307696313, -282.4663591245457042, -331.4445557061848717 ) ) ;
#37423=CARTESIAN_POINT ( 'NONE',  ( -37.11558689573416103, -277.9905979907121036, -347.1385107681607565 ) ) ;
#37425=CARTESIAN_POINT ( 'NONE',  ( 37.53464399305568833, -276.8866896574489260, -255.6559880793029436 ) ) ;
#37426=CARTESIAN_POINT ( 'NONE',  ( 30.91033621190086578, -284.2662352645559167, -285.9065529553535612 ) ) ;
#37429=CARTESIAN_POINT ( 'NONE',  ( -72.62788948468970318, -299.5851584109141754, -204.1658256102697351 ) ) ;
#37430=CARTESIAN_POINT ( 'NONE',  ( -34.86053410962789911, -293.1637250275788915, -197.0940046946069515 ) ) ;
#37431=CARTESIAN_POINT ( 'NONE',  ( -39.22395163547692931, -275.0960027690621246, -344.9821869586905336 ) ) ;
#37432=CARTESIAN_POINT ( 'NONE',  ( -20.69626094271407979, -290.6015799094691943, -344.5561741243666347 ) ) ;
#37433=CARTESIAN_POINT ( 'NONE',  ( 2.302737598095225824, -291.9469556524445579, -208.8828204492067186 ) ) ;
#37434=CARTESIAN_POINT ( 'NONE',  ( 28.84760934183840320, -287.5712474710974220, -309.5848635329697913 ) ) ;
#37436=CARTESIAN_POINT ( 'NONE',  ( -106.3053458097900545, -283.2990620952488712, -244.0845887565276371 ) ) ;
#37437=CARTESIAN_POINT ( 'NONE',  ( -110.7883500286502994, -282.9532948857978454, -276.3858478210781868 ) ) ;
#37439=CARTESIAN_POINT ( 'NONE',  ( -34.30963654725553624, -281.4062089212936826, -196.9179096800454545 ) ) ;
#37440=CARTESIAN_POINT ( 'NONE',  ( -103.5892900021988225, -290.9858905439799059, -309.2486624744716437 ) ) ;
#37441=CARTESIAN_POINT ( 'NONE',  ( -110.0280072607155120, -279.1483716307774898, -262.4806057647502371 ) ) ;
#37442=CARTESIAN_POINT ( 'NONE',  ( -6.035099822276707826, -291.2494487402477716, -200.4333443729489659 ) ) ;
#37443=CARTESIAN_POINT ( 'NONE',  ( 35.69234767254293672, -288.0520029906149944, -246.3124450938470034 ) ) ;
#37444=CARTESIAN_POINT ( 'NONE',  ( 32.65343452309119243, -287.6344093156233725, -238.2921932989166862 ) ) ;
#37445=CARTESIAN_POINT ( 'NONE',  ( -102.2393619153125144, -285.1732299390026810, -236.9351774717262060 ) ) ;
#37448=CARTESIAN_POINT ( 'NONE',  ( -70.38082524794387496, -293.4817050468574280, -202.1795831189753869 ) ) ;
#37449=CARTESIAN_POINT ( 'NONE',  ( -27.82588600098905118, -293.6186922873910703, -346.3268312306767598 ) ) ;
#37450=CARTESIAN_POINT ( 'NONE',  ( -8.657531191722618757, -275.7260967845510891, -337.7588768899171896 ) ) ;
#37451=CARTESIAN_POINT ( 'NONE',  ( -80.56086804385851963, -296.8318437976121800, -206.6935125192828480 ) ) ;
#37452=CARTESIAN_POINT ( 'NONE',  ( 23.16819565115745405, -291.4510493263329067, -228.2763003371824766 ) ) ;
#37453=CARTESIAN_POINT ( 'NONE',  ( -109.8823183692600907, -294.6000381193005637, -285.1155726733708775 ) ) ;
#37454=CARTESIAN_POINT ( 'NONE',  ( 2.442912765373550510, -293.8031455063644444, -208.6217891557181474 ) ) ;
#37455=CARTESIAN_POINT ( 'NONE',  ( 31.11214059008991129, -294.2829109717696952, -244.1256884269543264 ) ) ;
#37457=CARTESIAN_POINT ( 'NONE',  ( -70.03408964624055955, -293.4815471591751930, -338.0601135973089413 ) ) ;
#37458=CARTESIAN_POINT ( 'NONE',  ( -110.6383152259951714, -298.3474752891375488, -286.3140909482042957 ) ) ;
#37459=CARTESIAN_POINT ( 'NONE',  ( -37.25574734936045473, -289.9923039856906826, -343.5963626472061492 ) ) ;
#37460=CARTESIAN_POINT ( 'NONE',  ( 6.078919257242056062, -294.7781340909078835, -329.1330549387660653 ) ) ;
#37461=CARTESIAN_POINT ( 'NONE',  ( -105.9326596929985698, -280.9410224564196028, -239.0314339285689584 ) ) ;
#37462=CARTESIAN_POINT ( 'NONE',  ( -92.70524414728711804, -277.9642826135986979, -217.4822590635860422 ) ) ;
#37464=CARTESIAN_POINT ( 'NONE',  ( -34.09918009706371578, -273.4405203420124622, -193.5314436979977302 ) ) ;
#37465=CARTESIAN_POINT ( 'NONE',  ( 21.30055889832789617, -280.2658364039197636, -316.2130498709144035 ) ) ;
#37466=CARTESIAN_POINT ( 'NONE',  ( -53.57002169826647275, -278.2473137609144374, -195.8552417591963035 ) ) ;
#37467=CARTESIAN_POINT ( 'NONE',  ( -105.7400412630732518, -276.9616102279749157, -239.0638665336492750 ) ) ;
#37468=CARTESIAN_POINT ( 'NONE',  ( -109.1055128195557700, -271.3400360307750248, -254.0721613814322950 ) ) ;
#37469=DIRECTION ( 'NONE',  ( 0.000000000000000000, 0.000000000000000000, -1.000000000000000000 ) ) ;
#37471=CARTESIAN_POINT ( 'NONE',  ( -110.9638905495010874, -288.3669261625742024, -286.4290949801811621 ) ) ;
#37472=CARTESIAN_POINT ( 'NONE',  ( -114.0068376344051018, -290.6487534309579246, -262.6369593465452681 ) ) ;
#37473=CARTESIAN_POINT ( 'NONE',  ( -38.35877714513877379, -276.0395859228228232, -195.2013283002371793 ) ) ;
#37474=CARTESIAN_POINT ( 'NONE',  ( -67.53628947469199773, -295.6549983629083727, -201.8758242723695844 ) ) ;
#37475=CARTESIAN_POINT ( 'NONE',  ( -101.2904462688696725, -283.1863939766353155, -313.0560977462169490 ) ) ;
#37477=CARTESIAN_POINT ( 'NONE',  ( 34.95251751390191686, -279.8093045300353765, -290.3720257522728616 ) ) ;
#37478=DIRECTION ( 'NONE',  ( -1.000000000000000000, -0.000000000000000000, -0.000000000000000000 ) ) ;
#37479=CARTESIAN_POINT ( 'NONE',  ( 25.19418736623600097, -291.8191474391782094, -231.8407379668302326 ) ) ;
#37480=CARTESIAN_POINT ( 'NONE',  ( -71.72971496733919139, -283.7322233382939203, -204.5710737661032965 ) ) ;
#37482=CARTESIAN_POINT ( 'NONE',  ( 82.68040262957964615, -297.0801184085799491, -195.3611179825600175 ) ) ;
#37483=CARTESIAN_POINT ( 'NONE',  ( 32.70516106426969571, -291.2035751602908817, -243.5574263739953551 ) ) ;
#37484=CARTESIAN_POINT ( 'NONE',  ( -69.58271295524120603, -279.0838550669636220, -336.7600244727085510 ) ) ;
#37485=CARTESIAN_POINT ( 'NONE',  ( -55.59263170166233436, -284.4870809741044013, -344.7581086082990396 ) ) ;
#37486=CARTESIAN_POINT ( 'NONE',  ( -4.430786967408551824, -272.5622822969111212, -202.3308065067057271 ) ) ;
#37487=CARTESIAN_POINT ( 'NONE',  ( -52.08893400525370510, -285.8580710583424320, -198.8662294032218369 ) ) ;
#37488=CARTESIAN_POINT ( 'NONE',  ( 35.60219635229639579, -276.8501768434589962, -260.6367731040798503 ) ) ;
#37489=CARTESIAN_POINT ( 'NONE',  ( -51.30170664368912981, -278.0380690717825019, -342.1783857148822108 ) ) ;
#37490=CARTESIAN_POINT ( 'NONE',  ( -91.95719958110348102, -285.8317855447812121, -321.7817660464956475 ) ) ;
#37494=CARTESIAN_POINT ( 'NONE',  ( -68.22812767807562295, -295.2800603224667384, -340.8950006044734096 ) ) ;
#37495=CARTESIAN_POINT ( 'NONE',  ( -35.92701835163976654, -288.0498750724642036, -195.7297205570683616 ) ) ;
#37497=CARTESIAN_POINT ( 'NONE',  ( -88.52914483777347243, -293.1952119285919025, -334.4957818155094174 ) ) ;
#37498=CARTESIAN_POINT ( 'NONE',  ( -79.72844130231119664, -278.4143771956909177, -206.3845385109265180 ) ) ;
#37499=CARTESIAN_POINT ( 'NONE',  ( -97.70193146623168445, -289.5794152206813123, -223.8310577723109702 ) ) ;
#37500=CARTESIAN_POINT ( 'NONE',  ( -108.7604235962452037, -285.8347357563053492, -288.5290483093402827 ) ) ;
#37501=CARTESIAN_POINT ( 'NONE',  ( -94.74039640288346220, -280.9646091686304885, -223.6346406665721531 ) ) ;
#37502=CARTESIAN_POINT ( 'NONE',  ( 36.57903236361585186, -289.2214678645232198, -289.7087690605700345 ) ) ;
#37503=CARTESIAN_POINT ( 'NONE',  ( 4.527285024688798565, -284.4878019337590445, -332.6492585765331569 ) ) ;
#37504=CARTESIAN_POINT ( 'NONE',  ( 1.048875562918027970, -276.7215340536763506, -337.1686097628556809 ) ) ;
#37505=CARTESIAN_POINT ( 'NONE',  ( -97.74651051932343648, -271.1564459011171948, -226.1016842667979176 ) ) ;
#37506=CARTESIAN_POINT ( 'NONE',  ( -112.4012560575572905, -278.6003003003949061, -253.1837180568203394 ) ) ;
#37507=CARTESIAN_POINT ( 'NONE',  ( -55.67144113608279810, -299.7346915498959561, -198.1597643774171900 ) ) ;
#37509=CARTESIAN_POINT ( 'NONE',  ( 31.98288692825981272, -284.4805209788416960, -303.7098442033569654 ) ) ;
#37510=CARTESIAN_POINT ( 'NONE',  ( 11.15640338229844275, -272.9526403292505847, -211.7956515749848165 ) ) ;
#37512=CARTESIAN_POINT ( 'NONE',  ( -109.1914814245206173, -278.2344627587875721, -257.1098022196482020 ) ) ;
#37513=CARTESIAN_POINT ( 'NONE',  ( 36.50694323011791198, -277.0141089910986807, -290.7665520423612406 ) ) ;
#37514=CARTESIAN_POINT ( 'NONE',  ( -113.6711810870028359, -283.5085031039642445, -278.5238717547131841 ) ) ;
#37515=CARTESIAN_POINT ( 'NONE',  ( -26.30190637799861264, -290.6700151387158257, -343.5982377934620331 ) ) ;
#37516=CARTESIAN_POINT ( 'NONE',  ( -15.08150901362087204, -299.8461792891959590, -194.0488100198521693 ) ) ;
#37517=CARTESIAN_POINT ( 'NONE',  ( -112.7509503946451872, -297.9265635157346424, -256.8906431035279638 ) ) ;
#37518=CARTESIAN_POINT ( 'NONE',  ( -38.96218905668040122, -294.0319303719762729, -195.5453278999278268 ) ) ;
#37519=CARTESIAN_POINT ( 'NONE',  ( 15.19405727760773495, -280.3087349704866256, -323.7259149928286774 ) ) ;
#37520=CARTESIAN_POINT ( 'NONE',  ( 1.489159096981346408, -272.5939989760689741, -206.6115205403624770 ) ) ;
#37521=CARTESIAN_POINT ( 'NONE',  ( -108.5480278508402705, -285.8035598545636162, -297.6391946151897514 ) ) ;
#37522=CARTESIAN_POINT ( 'NONE',  ( -88.88814336202254651, -288.7177959898705240, -322.4877931423029054 ) ) ;
#37523=CARTESIAN_POINT ( 'NONE',  ( -112.5291768906040630, -274.3922002906971898, -284.1740904352106440 ) ) ;
#37525=CARTESIAN_POINT ( 'NONE',  ( 36.56981266951201803, -286.3713841404104414, -289.7439601455833440 ) ) ;
#37526=CARTESIAN_POINT ( 'NONE',  ( -31.87400628591920082, -288.6481172002576727, -343.2279066006028643 ) ) ;
#37528=CARTESIAN_POINT ( 'NONE',  ( -113.5142202591188720, -285.7435972221371117, -261.4594503700303108 ) ) ;
#37529=CARTESIAN_POINT ( 'NONE',  ( 32.11960236385683487, -276.1841455350033243, -292.8825509497615940 ) ) ;
#37530=CARTESIAN_POINT ( 'NONE',  ( -8.614199152875432475, -291.3397673769372318, -199.2539931800049260 ) ) ;
#37531=CARTESIAN_POINT ( 'NONE',  ( 34.49524211914257421, -282.5513700882429475, -297.7977087862402072 ) ) ;
#37533=CARTESIAN_POINT ( 'NONE',  ( 35.50797613771576522, -282.7844060178347263, -247.6535769292032967 ) ) ;
#37534=CARTESIAN_POINT ( 'NONE',  ( 13.66995374275020936, -282.6938633923983275, -328.0823601178042850 ) ) ;
#37535=CARTESIAN_POINT ( 'NONE',  ( -3.142946668124080745, -280.8502914417632610, -205.8292431900194117 ) ) ;
#37536=CARTESIAN_POINT ( 'NONE',  ( -82.08285599513421005, -294.9094976428775681, -214.2051214447836571 ) ) ;
#37537=CARTESIAN_POINT ( 'NONE',  ( 200.3681379904781465, 289.3007429391860228, -97.55793450621084162 ) ) ;
#37539=CARTESIAN_POINT ( 'NONE',  ( -110.8391933014092245, -280.3702994153910595, -284.5051734269482040 ) ) ;
#37540=CARTESIAN_POINT ( 'NONE',  ( 83.59802325294344882, 83.57088953122406849, -301.7212683633755432 ) ) ;
#37541=CARTESIAN_POINT ( 'NONE',  ( -89.82948962184238439, -228.9372499028087304, -344.6302353727376158 ) ) ;
#37542=CARTESIAN_POINT ( 'NONE',  ( -110.4760564755729746, -295.9223227184746747, -268.7223453535407884 ) ) ;
#37543=CARTESIAN_POINT ( 'NONE',  ( 36.22997111948400573, -292.7769263796104724, -247.8503185055625693 ) ) ;
#37544=CARTESIAN_POINT ( 'NONE',  ( 161.3931422174006514, 217.5860020225172491, -202.5160790841660514 ) ) ;
#37545=CARTESIAN_POINT ( 'NONE',  ( -20.65166408309490365, -296.8319791780506876, -193.9542942158973631 ) ) ;
#37546=CARTESIAN_POINT ( 'NONE',  ( -40.00720749556981559, -287.4859398097393637, -344.1630921471895022 ) ) ;
#37547=CARTESIAN_POINT ( 'NONE',  ( -102.5410590905519399, -297.9361215806902692, -305.8563158083793496 ) ) ;
#37548=CARTESIAN_POINT ( 'NONE',  ( -57.54593055370612120, -287.1011297558742967, -199.6467516099031343 ) ) ;
#37550=CARTESIAN_POINT ( 'NONE',  ( -13.84264205821067506, -295.6957170467346145, -343.4406259332304217 ) ) ;
#37551=CARTESIAN_POINT ( 'NONE',  ( -77.08779614944982939, -285.9963523650653201, -208.9966326678652706 ) ) ;
#37552=CARTESIAN_POINT ( 'NONE',  ( -37.59088967158061934, -296.8440274397970597, -193.7585943611897221 ) ) ;
#37553=CARTESIAN_POINT ( 'NONE',  ( -7.262855828185701412, -293.2395587303224147, -199.6402367457031062 ) ) ;
#37554=CARTESIAN_POINT ( 'NONE',  ( 23.98372463674631661, -294.6639772559295807, -316.8231366738565953 ) ) ;
#37555=CARTESIAN_POINT ( 'NONE',  ( -67.80312578678240243, -291.8075635755508870, -204.0065849163114251 ) ) ;
#37558=CARTESIAN_POINT ( 'NONE',  ( -78.08602790601095478, -275.4291078910717374, -206.7276837630186321 ) ) ;
#37559=CARTESIAN_POINT ( 'NONE',  ( -2.723187585705332037, -273.2944696992763625, -202.0122574492627052 ) ) ;
#37562=CARTESIAN_POINT ( 'NONE',  ( -89.17528491032298632, -277.2661824618260766, -327.2188913447552068 ) ) ;
#37564=CARTESIAN_POINT ( 'NONE',  ( -36.45371137686723984, -296.5433422393704745, -196.6680143152582048 ) ) ;
#37565=CARTESIAN_POINT ( 'NONE',  ( -21.41065430713900497, -274.9854101818856975, -342.9196221950773520 ) ) ;
#37566=CARTESIAN_POINT ( 'NONE',  ( -94.86377687975156903, -274.2704227116444144, -224.9140414991398984 ) ) ;
#37567=CARTESIAN_POINT ( 'NONE',  ( -104.6005375515376272, -273.8830666450586477, -241.2557143445264956 ) ) ;
#37568=CARTESIAN_POINT ( 'NONE',  ( -111.4599002293362702, -274.5245255676214811, -253.6139859404296715 ) ) ;
#37570=CARTESIAN_POINT ( 'NONE',  ( 10.75566765627312726, -272.7329247175058526, -212.2842431649167168 ) ) ;
#37571=CARTESIAN_POINT ( 'NONE',  ( -97.26218134082830602, -296.6204925839485895, -312.2350788598213285 ) ) ;
#37572=CARTESIAN_POINT ( 'NONE',  ( 33.68064685724496599, -292.3799151794447084, -289.6755657358717144 ) ) ;
#37574=CARTESIAN_POINT ( 'NONE',  ( -41.37494481440511152, -277.5939710936997926, -347.2069905948220025 ) ) ;
#37575=CARTESIAN_POINT ( 'NONE',  ( 35.60205065226340793, -275.7709323924987075, -274.3105143076345485 ) ) ;
#37576=CARTESIAN_POINT ( 'NONE',  ( -105.3534839891285060, -282.7811752266095482, -305.5152443238438877 ) ) ;
#37577=CARTESIAN_POINT ( 'NONE',  ( -97.63743886441584152, -299.1640323921772051, -225.4569763027148781 ) ) ;
#37579=CARTESIAN_POINT ( 'NONE',  ( -8.181212030536782365, -285.6412765830118019, -203.2621786373384509 ) ) ;
#37580=CARTESIAN_POINT ( 'NONE',  ( -83.65810834634042692, -275.9371548799731499, -328.1571939332554280 ) ) ;
#37581=CARTESIAN_POINT ( 'NONE',  ( -99.68384909428412755, -276.5901503890083859, -309.5566113658804852 ) ) ;
#37582=CARTESIAN_POINT ( 'NONE',  ( 26.96455796263020588, -283.0343519342358150, -231.6655152765091827 ) ) ;
#37583=CARTESIAN_POINT ( 'NONE',  ( 28.20906473603430697, -276.3115109789105190, -237.3425212625459437 ) ) ;
#37585=CARTESIAN_POINT ( 'NONE',  ( 37.43763592253894501, -273.7669438095991268, -255.7155958976435386 ) ) ;
#37586=CARTESIAN_POINT ( 'NONE',  ( -98.76589622790213241, -281.1395390408788444, -227.0356455514520349 ) ) ;
#37588=CARTESIAN_POINT ( 'NONE',  ( 8.909657572472564624, -288.6012342047308152, -210.6105857170054776 ) ) ;
#37589=CARTESIAN_POINT ( 'NONE',  ( -98.34275362693919931, -287.9582406316378638, -314.0163152306072334 ) ) ;
#37591=CARTESIAN_POINT ( 'NONE',  ( -108.4126790972154453, -271.4847261399625609, -251.4535893715823534 ) ) ;
#37592=CARTESIAN_POINT ( 'NONE',  ( -108.1371321504643959, -288.3985911579586627, -292.8667624560513900 ) ) ;
#37593=CARTESIAN_POINT ( 'NONE',  ( 197.9738562182569694, 296.4636489450776367, -54.00000000000000711 ) ) ;
#37595=CARTESIAN_POINT ( 'NONE',  ( 37.98733281522758887, -286.1897379819343996, -282.8574360961315506 ) ) ;
#37596=CARTESIAN_POINT ( 'NONE',  ( -53.84900324873385813, -284.8675625642646310, -342.3439394815155197 ) ) ;
#37597=CARTESIAN_POINT ( 'NONE',  ( -104.5255380858709344, -283.2577979975578160, -234.7477315733243870 ) ) ;
#37598=CARTESIAN_POINT ( 'NONE',  ( -101.1236770562101981, -291.0389213455058552, -234.7487109493455932 ) ) ;
#37599=CARTESIAN_POINT ( 'NONE',  ( 19.27792113855783285, -282.3158793617697597, -223.3352547110860655 ) ) ;
#37600=CARTESIAN_POINT ( 'NONE',  ( 15.95048526883005557, -283.0756710360772672, -320.5595098475272948 ) ) ;
#37601=CARTESIAN_POINT ( 'NONE',  ( -111.5098345817626040, -292.3608566650248690, -283.7565790884347052 ) ) ;
#37602=CARTESIAN_POINT ( 'NONE',  ( -34.04909031562004884, -298.2589888633038413, -193.3610277050512707 ) ) ;
#37603=CARTESIAN_POINT ( 'NONE',  ( 4.734782201528179968, -286.5685885933644954, -333.1216456320078123 ) ) ;
#37604=CARTESIAN_POINT ( 'NONE',  ( 33.01976959949786306, -275.9513472451616849, -301.6383233848166583 ) ) ;
#37605=CARTESIAN_POINT ( 'NONE',  ( -47.23691339035758574, -293.9057003455085919, -196.3750952792245528 ) ) ;
#37607=CARTESIAN_POINT ( 'NONE',  ( -106.6662871844225293, -287.4805209788416391, -237.0123917617630980 ) ) ;
#37608=CARTESIAN_POINT ( 'NONE',  ( -32.12731403894525073, -281.6698216102062133, -343.6690551796345403 ) ) ;
#37609=CARTESIAN_POINT ( 'NONE',  ( -105.9143137401185442, -276.1477636336859405, -301.2746351304886048 ) ) ;
#37612=CARTESIAN_POINT ( 'NONE',  ( -105.7857231747956916, -295.3866671249630826, -236.8669972660001406 ) ) ;
#37613=CARTESIAN_POINT ( 'NONE',  ( 35.68928468134305376, -274.8451466765188798, -266.1413440818419076 ) ) ;
#37614=CARTESIAN_POINT ( 'NONE',  ( -104.1933360997721394, -292.4869027017095959, -239.3519819349652948 ) ) ;
#37615=CARTESIAN_POINT ( 'NONE',  ( -69.13054301742045027, -292.5647597207795343, -204.3709258588713737 ) ) ;
#37616=CARTESIAN_POINT ( 'NONE',  ( -109.0698126027523926, -286.0747161948644361, -288.6108274780153806 ) ) ;
#37617=CARTESIAN_POINT ( 'NONE',  ( 37.78132488123052468, -295.1543623217763752, -284.4010640732971638 ) ) ;
#37618=CARTESIAN_POINT ( 'NONE',  ( 22.71049668625461848, -294.2289691711235946, -222.9373213547489456 ) ) ;
#37619=CARTESIAN_POINT ( 'NONE',  ( -109.3632621996024881, -296.2283329583613067, -282.2730700179022847 ) ) ;
#37620=CARTESIAN_POINT ( 'NONE',  ( 9.241551642968731883, -290.4123875611823564, -329.1403770801458677 ) ) ;
#37621=CARTESIAN_POINT ( 'NONE',  ( -90.43660223440669199, -283.9454276347947825, -326.2009835950146908 ) ) ;
#37622=CARTESIAN_POINT ( 'NONE',  ( -45.94125219169887231, -296.0237547665257125, -195.2920704253969859 ) ) ;
#37623=CARTESIAN_POINT ( 'NONE',  ( -101.4203214609275108, -283.8224439033913313, -313.1525799021392231 ) ) ;
#37624=CARTESIAN_POINT ( 'NONE',  ( -51.57026404567798039, -279.2149392249379503, -343.6372721431823152 ) ) ;
#37626=CARTESIAN_POINT ( 'NONE',  ( -110.7878736959665105, -283.3400389017655812, -270.8969657661165229 ) ) ;
#37628=CARTESIAN_POINT ( 'NONE',  ( 6.737930832372755141, -286.4529149418784186, -331.1045233509693162 ) ) ;
#37629=CARTESIAN_POINT ( 'NONE',  ( -85.99312505032125387, -277.5262283533841128, -212.2122561871963171 ) ) ;
#37630=CARTESIAN_POINT ( 'NONE',  ( -53.17117378510891967, -153.5335516589311737, -364.2630158522994179 ) ) ;
#37631=CARTESIAN_POINT ( 'NONE',  ( -110.3805893628636881, -284.0166549049548053, -273.6346452700706777 ) ) ;
#37632=CARTESIAN_POINT ( 'NONE',  ( 8.297596240448868343, -281.8659182009773190, -208.7723215107029091 ) ) ;
#37633=CARTESIAN_POINT ( 'NONE',  ( -41.75903509417830861, -288.1652468606594084, -347.0118059888877724 ) ) ;
#37634=CARTESIAN_POINT ( 'NONE',  ( -23.06855666265645510, -278.4727810662645311, -345.2660467195866545 ) ) ;
#37635=CARTESIAN_POINT ( 'NONE',  ( -34.29386784849671699, -278.3297499137577802, -346.8072362108209745 ) ) ;
#37636=CARTESIAN_POINT ( 'NONE',  ( -62.30695293087269704, -279.5516311147617898, -201.7093929148592224 ) ) ;
#37637=CARTESIAN_POINT ( 'NONE',  ( -49.16017066696437610, -275.8808498938869889, -196.6055294434982272 ) ) ;
#37638=CARTESIAN_POINT ( 'NONE',  ( 25.07699264894857905, -284.9922498286451287, -228.9885039889509812 ) ) ;
#37639=CARTESIAN_POINT ( 'NONE',  ( -82.36340345759107606, -291.2555654027345895, -331.8386475591551630 ) ) ;
#37640=CARTESIAN_POINT ( 'NONE',  ( -39.71275232492541107, -294.0029185774877192, -343.6443603086365783 ) ) ;
#37641=VERTEX_POINT ( 'NONE', #28888 ) ;
#37642=CARTESIAN_POINT ( 'NONE',  ( 34.08737187044444994, -293.4196534637811169, -285.5860100850539993 ) ) ;
#37643=CARTESIAN_POINT ( 'NONE',  ( -56.12643432226993667, -292.8954854425140866, -195.9516550952625096 ) ) ;
#37644=CARTESIAN_POINT ( 'NONE',  ( 34.43274187487774185, -282.0200121692074049, -256.4271846446987979 ) ) ;
#37645=CARTESIAN_POINT ( 'NONE',  ( -30.50496736591661318, -297.0561975967531794, -193.6714471065133978 ) ) ;
#37646=CARTESIAN_POINT ( 'NONE',  ( 18.27203574674027209, -287.4756648982031493, -217.1766575721160848 ) ) ;
#37648=CARTESIAN_POINT ( 'NONE',  ( -68.04154480222608470, -289.7776306228537919, -340.9533543019367130 ) ) ;
#37649=CARTESIAN_POINT ( 'NONE',  ( 2.454985290050144986, -286.9352139954348218, -209.1376640089450518 ) ) ;
#37651=CARTESIAN_POINT ( 'NONE',  ( -84.92324064171599218, -218.1701808897174715, -350.4119417867636344 ) ) ;
#37652=CARTESIAN_POINT ( 'NONE',  ( 192.6544724140480582, 276.0552902512551441, -124.0055601186182059 ) ) ;
#37653=CARTESIAN_POINT ( 'NONE',  ( -76.45075835905313966, -276.7867205270100612, -332.2517913679837989 ) ) ;
#37654=CARTESIAN_POINT ( 'NONE',  ( -97.91194419254118486, -276.9003649770493212, -311.6584739244761977 ) ) ;
#37655=CARTESIAN_POINT ( 'NONE',  ( -97.79382389457855140, -272.8564731349133012, -222.7031173553139638 ) ) ;
#37656=CARTESIAN_POINT ( 'NONE',  ( 186.2046704664805929, 260.4489007258302991, -151.5571721899337376 ) ) ;
#37657=CARTESIAN_POINT ( 'NONE',  ( -68.82782541750671612, -276.1423109118917409, -340.1029172073166933 ) ) ;
#37658=CARTESIAN_POINT ( 'NONE',  ( -76.54002866929528182, -297.3286924278899050, -335.5181367140972952 ) ) ;
#37659=CARTESIAN_POINT ( 'NONE',  ( -38.90517695359586980, -292.5243609972285412, -197.3163099394028279 ) ) ;
#37660=CARTESIAN_POINT ( 'NONE',  ( -106.3727411092069133, -297.7892413564482581, -236.6139077118289151 ) ) ;
#37661=CARTESIAN_POINT ( 'NONE',  ( -21.03610659092324653, -287.5233325544106151, -342.0226215668388363 ) ) ;
#37662=CARTESIAN_POINT ( 'NONE',  ( -97.73816644073109217, -273.8410081171123807, -222.7630125149007654 ) ) ;
#37663=CARTESIAN_POINT ( 'NONE',  ( -106.8686205551998540, -296.4218318016476701, -292.7735055452791926 ) ) ;
#37666=CARTESIAN_POINT ( 'NONE',  ( -111.0737817670128038, -280.2617639320028502, -286.8806318921927527 ) ) ;
#37667=EDGE_CURVE ( 'NONE', #58191, #57853, #26288, .T. ) ;
#37668=CARTESIAN_POINT ( 'NONE',  ( -95.04264424169875269, -280.2668934386103388, -225.1211432287273908 ) ) ;
#37669=CARTESIAN_POINT ( 'NONE',  ( -77.26319644249774399, -279.3393431236303286, -335.0770921082039990 ) ) ;
#37670=CARTESIAN_POINT ( 'NONE',  ( -72.21893659852504754, -272.0622194876918343, -205.3867320333394275 ) ) ;
#37673=CARTESIAN_POINT ( 'NONE',  ( 21.32770764968728017, -281.1095361591715118, -226.9016110156684363 ) ) ;
#37674=CARTESIAN_POINT ( 'NONE',  ( 5.789108410471958344, -277.2864156108663565, -333.9527225772035308 ) ) ;
#37675=CARTESIAN_POINT ( 'NONE',  ( 35.30794059788363626, -277.7916533601141964, -288.9898687286022323 ) ) ;
#37676=CARTESIAN_POINT ( 'NONE',  ( -90.92885079171797713, -276.3691525625011423, -324.9056232648151195 ) ) ;
#37679=CARTESIAN_POINT ( 'NONE',  ( 38.06438725825336178, -283.5263374061846662, -269.9143067520816999 ) ) ;
#37680=CARTESIAN_POINT ( 'NONE',  ( -12.19512293733743213, -291.5849070708507043, -201.6030324167746244 ) ) ;
#37682=CARTESIAN_POINT ( 'NONE',  ( 27.05693341984959233, -286.3479168327781963, -228.3357829610680199 ) ) ;
#37683=CARTESIAN_POINT ( 'NONE',  ( -64.44706033559685920, -281.6507206309740354, -339.2325450183386693 ) ) ;
#37684=CARTESIAN_POINT ( 'NONE',  ( 1.396174800651887260, -281.0986647465979331, -332.9885912476374301 ) ) ;
#37685=CARTESIAN_POINT ( 'NONE',  ( 5.575143043045670765, -284.7178221125593609, -209.4748501153949576 ) ) ;
#37687=CARTESIAN_POINT ( 'NONE',  ( -32.95453044752736105, -281.3137330514537666, -197.0952784151002959 ) ) ;
#37688=CARTESIAN_POINT ( 'NONE',  ( -111.5612411848370158, -270.6950922538807731, -259.2160366785121255 ) ) ;
#37689=CARTESIAN_POINT ( 'NONE',  ( 21.88842702488935643, -280.6018506554717646, -318.3215814268220925 ) ) ;
#37690=CARTESIAN_POINT ( 'NONE',  ( 33.60309272334027497, -295.8689257732274882, -294.8481270805441454 ) ) ;
#37691=CARTESIAN_POINT ( 'NONE',  ( -96.16207195449918288, -287.1941086603724216, -223.5616277089561947 ) ) ;
#37693=CARTESIAN_POINT ( 'NONE',  ( -74.00205074352921031, -293.4891656483618476, -204.2904520863180267 ) ) ;
#37694=CARTESIAN_POINT ( 'NONE',  ( 37.69952133095186753, -273.5684581228775301, -271.6439160306233589 ) ) ;
#37695=CARTESIAN_POINT ( 'NONE',  ( -46.01771493812130132, -288.3565515813159550, -346.7612723019060468 ) ) ;
#37696=CARTESIAN_POINT ( 'NONE',  ( 34.84588310033183234, -292.1530112701957478, -285.7641872428404781 ) ) ;
#37698=CARTESIAN_POINT ( 'NONE',  ( -108.3007510680304080, -276.9859520510550510, -289.4937228425025637 ) ) ;
#37699=CARTESIAN_POINT ( 'NONE',  ( -96.25511390437439729, -295.3168522175690782, -225.1732222194624740 ) ) ;
#37700=CARTESIAN_POINT ( 'NONE',  ( -66.50944301466391551, -290.7573771064948573, -337.8727843772070969 ) ) ;
#37703=CARTESIAN_POINT ( 'NONE',  ( 28.88359954126167750, -291.5350766291451805, -232.4544241809067273 ) ) ;
#37704=CARTESIAN_POINT ( 'NONE',  ( -14.33575256702261669, -287.9554799457537229, -200.1850115788404878 ) ) ;
#37705=CARTESIAN_POINT ( 'NONE',  ( -113.2402406540008002, -288.7456447905061054, -274.0197458076002590 ) ) ;
#37706=CARTESIAN_POINT ( 'NONE',  ( 36.26926440092935167, -288.9501699191234820, -268.2778148346371836 ) ) ;
#37708=CARTESIAN_POINT ( 'NONE',  ( 30.10667718276161864, -287.9739422950855214, -241.8870976369559571 ) ) ;
#37709=CARTESIAN_POINT ( 'NONE',  ( -63.66743565242112624, -297.3735375276176001, -340.9682171409212401 ) ) ;
#37711=CARTESIAN_POINT ( 'NONE',  ( -74.22260853141756343, -290.7362035837512622, -337.5162988473455812 ) ) ;
#37712=CARTESIAN_POINT ( 'NONE',  ( -35.35360162160101538, -278.0970711081669151, -195.0192884189522147 ) ) ;
#37713=CARTESIAN_POINT ( 'NONE',  ( -19.76517645851018301, -280.6053071016204967, -195.3609824881742441 ) ) ;
#37714=CARTESIAN_POINT ( 'NONE',  ( -82.22308794841831059, -279.1248546121124150, -207.8198890310584375 ) ) ;
#37715=CARTESIAN_POINT ( 'NONE',  ( -73.31142217984276499, -283.5750233019674624, -204.5348150507924174 ) ) ;
#37716=CARTESIAN_POINT ( 'NONE',  ( -111.5352550897782749, -274.3943000018521730, -270.3845729371874427 ) ) ;
#37717=CARTESIAN_POINT ( 'NONE',  ( -1.346756639984390436, -278.6745402880802658, -205.4363189856392182 ) ) ;
#37718=CARTESIAN_POINT ( 'NONE',  ( -57.96198189079880336, -281.3182150669873636, -342.5248510673511078 ) ) ;
#37720=CARTESIAN_POINT ( 'NONE',  ( -79.85610541683962538, -276.0952751281701012, -333.7906028290099698 ) ) ;
#37721=CARTESIAN_POINT ( 'NONE',  ( -82.38303917391709774, -298.9449961160740941, -211.9698892282532654 ) ) ;
#37722=CARTESIAN_POINT ( 'NONE',  ( -99.08715357158504844, -284.0802417515357092, -224.7875916228985886 ) ) ;
#37723=CARTESIAN_POINT ( 'NONE',  ( -110.5031764828875396, -273.3548555555994426, -270.3713160627550565 ) ) ;
#37724=CARTESIAN_POINT ( 'NONE',  ( -89.77185585563556458, -274.7552957348602831, -214.7039098860404067 ) ) ;
#37725=CARTESIAN_POINT ( 'NONE',  ( 30.19599232763608043, -274.8453020664975952, -242.4659859445256416 ) ) ;
#37726=CARTESIAN_POINT ( 'NONE',  ( -94.59304442827847481, -297.8818750939501001, -318.8297842443670902 ) ) ;
#37727=CARTESIAN_POINT ( 'NONE',  ( -95.45690778130091303, -290.0360474077004369, -320.8747066884077981 ) ) ;
#37728=CARTESIAN_POINT ( 'NONE',  ( -76.72077358112996137, -277.6096693091433281, -205.8133274144104234 ) ) ;
#37729=CARTESIAN_POINT ( 'NONE',  ( -95.45969724777727095, -289.7027411976405347, -320.8714972655885163 ) ) ;
#37730=CARTESIAN_POINT ( 'NONE',  ( -26.45170130298138744, -287.9690568858730444, -342.8334356260376126 ) ) ;
#37731=CARTESIAN_POINT ( 'NONE',  ( 37.71025294593471244, -291.5516736992122446, -270.3367095491944383 ) ) ;
#37734=CARTESIAN_POINT ( 'NONE',  ( -109.7602561260798808, -290.1922231692020091, -260.3144446255313937 ) ) ;
#37736=CARTESIAN_POINT ( 'NONE',  ( -40.81785317066410101, -286.9508117773478375, -193.6231241796697020 ) ) ;
#37737=CARTESIAN_POINT ( 'NONE',  ( -82.08285599513421005, -298.1948066931273615, -326.5171145203363494 ) ) ;
#37738=CARTESIAN_POINT ( 'NONE',  ( 13.23177851729148458, -293.4242757055536686, -328.1822876491806369 ) ) ;
#37739=CARTESIAN_POINT ( 'NONE',  ( -49.99534544201929975, -284.5254039480373649, -345.8678343240129607 ) ) ;
#37740=CARTESIAN_POINT ( 'NONE',  ( -52.08686027762424686, -285.6914178420956318, -198.8658016559107296 ) ) ;
#37741=CARTESIAN_POINT ( 'NONE',  ( 21.86862158560414571, -276.2614182090201211, -226.8251411176449608 ) ) ;
#37742=CARTESIAN_POINT ( 'NONE',  ( 31.37967797716864027, -291.1880930204496281, -241.0874106872614391 ) ) ;
#37743=CARTESIAN_POINT ( 'NONE',  ( -11.33524563461924828, -273.1934724416707923, -201.6715427892335413 ) ) ;
#37746=CARTESIAN_POINT ( 'NONE',  ( -3.241968658763197730, -294.2809074460785155, -339.3898654669944221 ) ) ;
#37747=CARTESIAN_POINT ( 'NONE',  ( -22.19016968178731020, -288.1677394615121557, -197.4264962426103693 ) ) ;
#37748=CARTESIAN_POINT ( 'NONE',  ( -97.99798081555323392, -298.2610521273613813, -223.4111628241926439 ) ) ;
#37749=CARTESIAN_POINT ( 'NONE',  ( 9.088851792067538682, -287.3608727325254222, -213.8978864400777411 ) ) ;
#37750=CARTESIAN_POINT ( 'NONE',  ( -113.8083720090882451, -277.7029385908161316, -263.0244537588394564 ) ) ;
#37751=CARTESIAN_POINT ( 'NONE',  ( 39.13661133486895949, -294.3101867204293285, -278.8753295318030041 ) ) ;
#37752=CARTESIAN_POINT ( 'NONE',  ( 27.82900540908005382, -286.2033991057485878, -309.0015711177097160 ) ) ;
#37754=CARTESIAN_POINT ( 'NONE',  ( 24.01469349679570797, -294.5049369647204003, -316.8491514209268871 ) ) ;
#37755=CARTESIAN_POINT ( 'NONE',  ( -87.94830204885226976, -291.6542034651085373, -217.6503829621510420 ) ) ;
#37757=CARTESIAN_POINT ( 'NONE',  ( 144.7857639756989272, -297.1570670221753971, -195.3611179825600175 ) ) ;
#37758=CARTESIAN_POINT ( 'NONE',  ( 85.24291059907943691, 81.26895831532213776, -298.9807373496020659 ) ) ;
#37760=CARTESIAN_POINT ( 'NONE',  ( 35.18394553432579386, -288.7691767095375894, -246.4701583390247492 ) ) ;
#37761=CARTESIAN_POINT ( 'NONE',  ( 13.79469577742117181, -279.9094976428775681, -334.5364918783848793 ) ) ;
#37763=CARTESIAN_POINT ( 'NONE',  ( -85.07341159308739975, -282.6498349985838558, -326.0020183466536992 ) ) ;
#37764=CARTESIAN_POINT ( 'NONE',  ( -112.7737633824739731, -278.0259807495030486, -285.7803694997610933 ) ) ;
#37765=CARTESIAN_POINT ( 'NONE',  ( 35.43902827600663841, -283.7770093004746172, -287.8224330372684108 ) ) ;
#37766=CARTESIAN_POINT ( 'NONE',  ( -111.0078494383391643, -273.9054044750961907, -284.0227232199477498 ) ) ;
#37767=CARTESIAN_POINT ( 'NONE',  ( -66.94390476819259561, -284.2464329214698751, -199.9174115631348343 ) ) ;
#37768=CARTESIAN_POINT ( 'NONE',  ( 26.36739446536032361, -285.0481796969785364, -231.4638421486721995 ) ) ;
#37769=CARTESIAN_POINT ( 'NONE',  ( -60.51620943829987453, -275.6152834882319098, -198.1728337017907506 ) ) ;
#37770=CARTESIAN_POINT ( 'NONE',  ( -101.2714380519233686, -297.5274888796026858, -234.9919640418008271 ) ) ;
#37771=CARTESIAN_POINT ( 'NONE',  ( -28.85555215543839225, -293.6272811269888052, -343.4140422409176381 ) ) ;
#37772=CARTESIAN_POINT ( 'NONE',  ( -112.0741474413762688, -278.9759411383659540, -288.5373421947147676 ) ) ;
#37773=CARTESIAN_POINT ( 'NONE',  ( 17.43522920221995776, -276.2413857850881982, -318.6343852935881387 ) ) ;
#37774=CARTESIAN_POINT ( 'NONE',  ( -23.42491818985267926, -299.1636407243324811, -193.5942472848419698 ) ) ;
#37775=CARTESIAN_POINT ( 'NONE',  ( -64.99649303227438679, -276.3252933695447950, -341.9483295330051078 ) ) ;
#37776=CARTESIAN_POINT ( 'NONE',  ( -100.2953508598967574, -247.7937573541214249, -334.1010632675480565 ) ) ;
#37777=CARTESIAN_POINT ( 'NONE',  ( -93.91613561194917281, -275.8684529495638458, -319.6178235012662299 ) ) ;
#37778=CARTESIAN_POINT ( 'NONE',  ( -113.7215832906442330, -298.0225411687098926, -266.7811269161292671 ) ) ;
#37779=CARTESIAN_POINT ( 'NONE',  ( -20.25526795762937127, -276.7662352645559167, -195.3538533559490702 ) ) ;
#37780=DIRECTION ( 'NONE',  ( -1.000000000000000000, -0.000000000000000000, -0.000000000000000000 ) ) ;
#37781=CARTESIAN_POINT ( 'NONE',  ( -56.38601138994710027, -284.3830813834740638, -341.1533511814076292 ) ) ;
#37782=CARTESIAN_POINT ( 'NONE',  ( -108.3479269349698342, -285.9635469242175532, -297.5647797368438319 ) ) ;
#37783=CARTESIAN_POINT ( 'NONE',  ( 30.05896838192226639, -286.5199305538867520, -241.9272974550434583 ) ) ;
#37784=CARTESIAN_POINT ( 'NONE',  ( -88.06584979592813056, -277.7283686652557435, -216.6854663963555083 ) ) ;
#37785=CARTESIAN_POINT ( 'NONE',  ( -108.5705212828705157, -286.1399632973974008, -291.3186634987029038 ) ) ;
#37786=CARTESIAN_POINT ( 'NONE',  ( -67.57318300133543687, -278.1280593844198279, -203.1405009579335967 ) ) ;
#37787=CARTESIAN_POINT ( 'NONE',  ( -72.98029933047352813, -278.6158898784741496, -334.4389367112646596 ) ) ;
#37789=CARTESIAN_POINT ( 'NONE',  ( -108.0012170349966567, -273.2919539880256821, -251.5869293900192076 ) ) ;
#37790=CARTESIAN_POINT ( 'NONE',  ( 37.82456592097646109, -282.1543792110126674, -254.3548339861530962 ) ) ;
#37791=CARTESIAN_POINT ( 'NONE',  ( 2.068005410463290339, -283.0316567554436915, -336.4398741192388798 ) ) ;
#37795=CARTESIAN_POINT ( 'NONE',  ( 30.59059424230705915, -289.8520486929858748, -304.0281190475556059 ) ) ;
#37796=CARTESIAN_POINT ( 'NONE',  ( -86.20055025551432948, -296.5505580921436604, -215.9054985227050167 ) ) ;
#37798=CARTESIAN_POINT ( 'NONE',  ( -72.11873837068029047, -290.9530080029579153, -201.7617707338883974 ) ) ;
#37799=CARTESIAN_POINT ( 'NONE',  ( 21.71764038975468836, -286.6449205678022167, -314.4583285992746369 ) ) ;
#37800=CARTESIAN_POINT ( 'NONE',  ( 6.178595397995848337, -287.0234379615165494, -329.7656499623095669 ) ) ;
#37801=CARTESIAN_POINT ( 'NONE',  ( -71.37589818712689294, -286.7972193673790002, -205.3318640405370843 ) ) ;
#37802=CARTESIAN_POINT ( 'NONE',  ( -94.63821083568684855, -275.8824393043251462, -318.7763050927415520 ) ) ;
#37803=CARTESIAN_POINT ( 'NONE',  ( -59.81102077776797898, -287.7383936417400037, -343.1729991793357044 ) ) ;
#37804=CARTESIAN_POINT ( 'NONE',  ( -29.69290381712577087, -288.1491791821498509, -195.7521603230860308 ) ) ;
#37805=CARTESIAN_POINT ( 'NONE',  ( -64.80158629606067677, -287.4096252032110783, -340.3874302961012859 ) ) ;
#37806=CARTESIAN_POINT ( 'NONE',  ( -10.87959983794257823, -283.6398546170017880, -338.7022512533970371 ) ) ;
#37807=CARTESIAN_POINT ( 'NONE',  ( -61.13304196143574387, -293.7442956288926439, -199.0041141731558128 ) ) ;
#37810=CARTESIAN_POINT ( 'NONE',  ( -65.03740017501561965, -299.6134254742047460, -200.0039601905290567 ) ) ;
#37811=CARTESIAN_POINT ( 'NONE',  ( -41.04916566346640394, -279.2014650675163239, -197.2936393989929797 ) ) ;
#37812=CARTESIAN_POINT ( 'NONE',  ( 16.71818628295263665, -278.8207651294118818, -218.3010416923969501 ) ) ;
#37813=CARTESIAN_POINT ( 'NONE',  ( 19.40351041030578827, -293.4558892461126902, -322.2472912541077221 ) ) ;
#37814=CARTESIAN_POINT ( 'NONE',  ( -52.78280127321203707, -296.2509912985147480, -198.1421037400120326 ) ) ;
#37815=CARTESIAN_POINT ( 'NONE',  ( 32.60663964426203165, -273.9665152204736387, -295.9772954130647804 ) ) ;
#37816=CARTESIAN_POINT ( 'NONE',  ( 4.108237434672163957, -295.7956527958423294, -331.0500473937844959 ) ) ;
#37818=CARTESIAN_POINT ( 'NONE',  ( -40.39297037167825977, -296.4944671830851348, -194.0638207371761439 ) ) ;
#37819=CARTESIAN_POINT ( 'NONE',  ( -112.9374056294798550, -294.6944509249191810, -278.0593854609253981 ) ) ;
#37820=CARTESIAN_POINT ( 'NONE',  ( 36.01322465072367862, -295.0542162284260144, -276.2288199817065788 ) ) ;
#37822=CARTESIAN_POINT ( 'NONE',  ( -94.06125868345739605, -296.7020844567787208, -316.5922034578405828 ) ) ;
#37825=CARTESIAN_POINT ( 'NONE',  ( -30.99667147627619812, -284.1520367043187321, -195.2605087894166900 ) ) ;
#37826=CARTESIAN_POINT ( 'NONE',  ( -110.3742624300891748, -296.5736311168014367, -268.7328962846926288 ) ) ;
#37827=CARTESIAN_POINT ( 'NONE',  ( -101.4191420572007871, -283.9890970573874256, -313.1543460418805580 ) ) ;
#37828=CARTESIAN_POINT ( 'NONE',  ( -9.416466136213701432, -282.3344519962977301, -200.1507519025080342 ) ) ;
#37829=CIRCLE ( 'NONE', #40780, 1.000000000000000888 ) ;
#37830=CARTESIAN_POINT ( 'NONE',  ( 5.171536239335461360, -286.2764926188042409, -206.1231063992670727 ) ) ;
#37831=CARTESIAN_POINT ( 'NONE',  ( -82.82360416465972719, -289.4288574986434810, -210.8697706112226626 ) ) ;
#37832=CARTESIAN_POINT ( 'NONE',  ( -85.28047601435908120, -276.9094976428775681, -210.1954327657594206 ) ) ;
#37833=CARTESIAN_POINT ( 'NONE',  ( 29.26390660990996651, -285.8203483262448117, -239.2976888795785442 ) ) ;
#37834=CARTESIAN_POINT ( 'NONE',  ( -111.9651210933101595, -289.2496862974836063, -288.1045637006901643 ) ) ;
#37836=CARTESIAN_POINT ( 'NONE',  ( -109.3682417825332465, -297.9424386252651971, -286.4427135188584543 ) ) ;
#37837=CARTESIAN_POINT ( 'NONE',  ( -98.11880804010954193, -280.5997480120203136, -224.0283581363119083 ) ) ;
#37838=CARTESIAN_POINT ( 'NONE',  ( 0.9122612509525566127, -292.5644924864690211, -335.2844669534731565 ) ) ;
#37839=CARTESIAN_POINT ( 'NONE',  ( 33.13510413581197867, -280.9659617420585960, -251.2054813130784510 ) ) ;
#37840=CARTESIAN_POINT ( 'NONE',  ( -44.79351154302201365, -295.3105474605857808, -347.0530951707714280 ) ) ;
#37841=CARTESIAN_POINT ( 'NONE',  ( -108.6107682297680270, -282.9546897511216912, -245.2606373344350459 ) ) ;
#37842=CARTESIAN_POINT ( 'NONE',  ( -105.6095004350705295, -280.9612874923071786, -239.1794537842767454 ) ) ;
#37843=CARTESIAN_POINT ( 'NONE',  ( -94.13258990755861078, -294.9582825502211563, -316.6215412285289403 ) ) ;
#37844=CARTESIAN_POINT ( 'NONE',  ( -92.77558565261395529, -271.2595425627999361, -219.5768502237933717 ) ) ;
#37847=CARTESIAN_POINT ( 'NONE',  ( 34.55023997769868771, -283.7916519174600580, -290.4458323788167604 ) ) ;
#37848=CARTESIAN_POINT ( 'NONE',  ( -109.7964231187581703, -296.1886927427498222, -260.5822927291129076 ) ) ;
#37850=CARTESIAN_POINT ( 'NONE',  ( -110.4683760289727132, -281.8380690714489560, -287.0191576251351080 ) ) ;
#37851=CARTESIAN_POINT ( 'NONE',  ( 28.36977180997978465, -274.2272177127116493, -230.4327391209765779 ) ) ;
#37854=CARTESIAN_POINT ( 'NONE',  ( 21.12306777744842989, -289.5363890634069435, -319.7085514306408527 ) ) ;
#37855=CARTESIAN_POINT ( 'NONE',  ( -72.62508707559196353, -291.4048058399475281, -206.3974875332536953 ) ) ;
#37856=CARTESIAN_POINT ( 'NONE',  ( -6.496721337991925971, -281.9848599690938613, -203.4198082974186832 ) ) ;
#37857=CARTESIAN_POINT ( 'NONE',  ( -59.73760420987919417, -275.3574279845327055, -199.9878846632465752 ) ) ;
#37858=CARTESIAN_POINT ( 'NONE',  ( -4.154371310788768312, -279.2947154676454602, -204.8816500456040899 ) ) ;
#37859=CARTESIAN_POINT ( 'NONE',  ( -18.49029900600233134, -278.8094562979103443, -342.9533029717113664 ) ) ;
#37861=CARTESIAN_POINT ( 'NONE',  ( -94.14382996827848160, -273.0927270366960329, -218.3559024421128072 ) ) ;
#37862=CARTESIAN_POINT ( 'NONE',  ( -32.07942449665793561, -294.0391766735301644, -196.0944767445531340 ) ) ;
#37865=CARTESIAN_POINT ( 'NONE',  ( 37.63316176299144900, -291.5485579843812047, -259.0961815992994843 ) ) ;
#37866=CARTESIAN_POINT ( 'NONE',  ( -96.32734431689104326, -272.6640155438018951, -227.1646356837109977 ) ) ;
#37868=CARTESIAN_POINT ( 'NONE',  ( 28.86439211801948446, -294.5748309556944378, -232.4208873458419191 ) ) ;
#37869=CARTESIAN_POINT ( 'NONE',  ( -54.49178911615187815, -282.3376638359844719, -195.3683826091709363 ) ) ;
#37870=CARTESIAN_POINT ( 'NONE',  ( -14.01819356607601463, -288.3554475995405824, -199.2009212967978158 ) ) ;
#37871=CARTESIAN_POINT ( 'NONE',  ( 4.129456990265810923, -274.4916737323193843, -332.6521410263596294 ) ) ;
#37872=CARTESIAN_POINT ( 'NONE',  ( 30.38624796905902059, -277.0623981502474749, -239.3457495839268745 ) ) ;
#37873=CARTESIAN_POINT ( 'NONE',  ( -11.74248024021450476, -290.4677657347916124, -200.4062835822410023 ) ) ;
#37874=CARTESIAN_POINT ( 'NONE',  ( -25.61058765086342248, -282.0605198663932356, -195.5100226104716796 ) ) ;
#37876=CARTESIAN_POINT ( 'NONE',  ( -58.98621574447633975, -282.6881675588109033, -340.2384550567359156 ) ) ;
#37877=CARTESIAN_POINT ( 'NONE',  ( -70.15622494353128502, -278.5540352753159254, -339.6914360324055906 ) ) ;
#37878=CARTESIAN_POINT ( 'NONE',  ( -74.09901423582336122, -282.3239683497937449, -337.6282586243166861 ) ) ;
#37879=CARTESIAN_POINT ( 'NONE',  ( -62.31807115371835692, -278.3103704656411423, -343.0051362575957228 ) ) ;
#37880=CARTESIAN_POINT ( 'NONE',  ( 25.50693952603189274, -277.6497980191384158, -313.7279578725210172 ) ) ;
#37882=CARTESIAN_POINT ( 'NONE',  ( -53.35057174420112602, -282.3376638359844151, -200.3683826091709648 ) ) ;
#37884=CARTESIAN_POINT ( 'NONE',  ( -112.2102538266806420, -298.6093062984550102, -265.9226144867148491 ) ) ;
#37885=CARTESIAN_POINT ( 'NONE',  ( -92.63585976976855818, -290.9477255737501764, -318.5699222785102052 ) ) ;
#37886=CARTESIAN_POINT ( 'NONE',  ( -98.24192166784143865, -275.9826242696316285, -313.5459242475561155 ) ) ;
#37887=CARTESIAN_POINT ( 'NONE',  ( -65.05626370705968498, -291.1693201541895064, -341.1689339508319563 ) ) ;
#37888=CARTESIAN_POINT ( 'NONE',  ( -34.84550506760024291, -291.4329202995482433, -197.3018155038428461 ) ) ;
#37889=CARTESIAN_POINT ( 'NONE',  ( 31.62947258698452302, -287.4996641502236230, -304.5767688223044161 ) ) ;
#37891=CARTESIAN_POINT ( 'NONE',  ( -105.9652657463868479, -282.5911136779089929, -297.6526102722045835 ) ) ;
#37892=CARTESIAN_POINT ( 'NONE',  ( -109.8644192410052653, -292.2062103438839245, -286.2732203357548428 ) ) ;
#37893=CARTESIAN_POINT ( 'NONE',  ( -110.5639283553350367, -282.9175442280081256, -279.1217415197455125 ) ) ;
#37894=CARTESIAN_POINT ( 'NONE',  ( 26.88172111737788228, -282.3820820374240270, -234.6316393914941898 ) ) ;
#37895=CARTESIAN_POINT ( 'NONE',  ( -112.6348559637020799, -291.3049127527841620, -285.3863339856826542 ) ) ;
#37896=CARTESIAN_POINT ( 'NONE',  ( -108.2302647728582770, -278.8106888934681820, -288.0988227970166236 ) ) ;
#37897=CARTESIAN_POINT ( 'NONE',  ( 22.80589254233456842, -291.7091276413913761, -222.9030792161684076 ) ) ;
#37898=CARTESIAN_POINT ( 'NONE',  ( -23.82438203873358873, -287.0233348401827698, -194.6668090308007493 ) ) ;
#37899=CARTESIAN_POINT ( 'NONE',  ( 28.64253936591920890, -287.5269053398747019, -230.6906288048405145 ) ) ;
#37900=CARTESIAN_POINT ( 'NONE',  ( -94.28367814786605550, -284.0730989365664527, -316.0604412714987461 ) ) ;
#37903=CARTESIAN_POINT ( 'NONE',  ( -50.37750192876276856, -293.7478386542660473, -195.7261841411425962 ) ) ;
#37904=CARTESIAN_POINT ( 'NONE',  ( -105.5258539099958028, -294.7859214051467802, -305.1797347298445402 ) ) ;
#37905=CARTESIAN_POINT ( 'NONE',  ( 21.01718239492835494, -275.2306949174555939, -314.6064485773082993 ) ) ;
#37906=CARTESIAN_POINT ( 'NONE',  ( -78.14134631940559927, -296.8673582020284698, -205.1790525265601275 ) ) ;
#37907=CARTESIAN_POINT ( 'NONE',  ( 17.58453420211446527, -292.7284540843510285, -319.5107442805134497 ) ) ;
#37908=CARTESIAN_POINT ( 'NONE',  ( -99.59764393805663474, -294.2445650762564355, -310.4821818053980564 ) ) ;
#37909=CARTESIAN_POINT ( 'NONE',  ( -108.4971888562050992, -291.9941278445810440, -252.3092113475963743 ) ) ;
#37910=CARTESIAN_POINT ( 'NONE',  ( 33.05082817476538537, -294.9020240355306441, -290.8786394097517132 ) ) ;
#37912=CARTESIAN_POINT ( 'NONE',  ( -32.16482345846244328, -292.9868597415327258, -345.3622451808073492 ) ) ;
#37913=CARTESIAN_POINT ( 'NONE',  ( -88.67267991231055646, -299.3324894279874684, -215.6086549289517222 ) ) ;
#37914=CARTESIAN_POINT ( 'NONE',  ( 3.756531542628308795, -289.4255022940145636, -331.0386396783659393 ) ) ;
#37915=CARTESIAN_POINT ( 'NONE',  ( 9.523272992201938791, -278.3916522198820758, -329.4369280531495292 ) ) ;
#37916=CARTESIAN_POINT ( 'NONE',  ( -104.3535256286225206, -277.7182137153757253, -233.4461682377362024 ) ) ;
#37917=CARTESIAN_POINT ( 'NONE',  ( -31.25984375472080856, -273.4756288010908065, -193.6906704887533692 ) ) ;
#37918=CARTESIAN_POINT ( 'NONE',  ( 19.95993369407761975, -278.9709942436958841, -222.8246241192646551 ) ) ;
#37919=CARTESIAN_POINT ( 'NONE',  ( -111.7081662790270116, -276.7420514374772438, -286.9764461759999676 ) ) ;
#37920=CARTESIAN_POINT ( 'NONE',  ( -90.77723647660442907, -294.5144331977039656, -320.8912095960502029 ) ) ;
#37921=CARTESIAN_POINT ( 'NONE',  ( -99.71146802823204780, -275.1163471905415463, -228.6157160029798945 ) ) ;
#37922=CARTESIAN_POINT ( 'NONE',  ( -29.98784991494091656, -274.7991011438192572, -197.6300135279857955 ) ) ;
#37923=DIRECTION ( 'NONE',  ( 3.961265963009670520E-15, 7.202301750926674102E-15, -1.000000000000000000 ) ) ;
#37924=CARTESIAN_POINT ( 'NONE',  ( -76.29691754400595016, -289.5546316110525709, -205.7959278483178025 ) ) ;
#37925=CARTESIAN_POINT ( 'NONE',  ( -113.8135556978273115, -290.4340524855738863, -279.8042728030280273 ) ) ;
#37926=CARTESIAN_POINT ( 'NONE',  ( 25.38624446038517135, -276.9943808511857242, -228.9457416828620637 ) ) ;
#37927=CARTESIAN_POINT ( 'NONE',  ( -112.2078474041528153, -294.5737924853900154, -268.6665875318754502 ) ) ;
#37928=CARTESIAN_POINT ( 'NONE',  ( -69.12900813159500046, -282.6568709926306724, -340.3306733251769174 ) ) ;
#37930=CARTESIAN_POINT ( 'NONE',  ( 18.51668205331070283, -280.2492099564546493, -320.4285477096707950 ) ) ;
#37932=CARTESIAN_POINT ( 'NONE',  ( -60.36906169767474495, -290.5418558152254036, -200.6165381951582845 ) ) ;
#37933=CARTESIAN_POINT ( 'NONE',  ( -108.5328522624296141, -282.9675988319892781, -249.1429434439755539 ) ) ;
#37936=CARTESIAN_POINT ( 'NONE',  ( 35.37921285071867317, -291.7876982231325087, -288.7096729066396392 ) ) ;
#37937=CARTESIAN_POINT ( 'NONE',  ( -101.2657006484102027, -279.6508405594983628, -307.3440872695285861 ) ) ;
#37938=CARTESIAN_POINT ( 'NONE',  ( -44.36743251959935463, -284.3440870560242502, -346.6942614041393540 ) ) ;
#37939=CARTESIAN_POINT ( 'NONE',  ( -35.53327204678248563, -272.1544973493340080, -194.8098739069588134 ) ) ;
#37940=CARTESIAN_POINT ( 'NONE',  ( -72.37401242321359973, -285.5748606903512155, -206.3020960892154676 ) ) ;
#37941=CARTESIAN_POINT ( 'NONE',  ( 7.957272456310147568, -277.8448265606603513, -328.4206999836026739 ) ) ;
#37942=CARTESIAN_POINT ( 'NONE',  ( 17.56316655420695128, -277.0440886599989199, -318.7334835776064779 ) ) ;
#37943=CARTESIAN_POINT ( 'NONE',  ( -82.65407103244992015, -285.6710795554912465, -330.1907914476502697 ) ) ;
#37946=CARTESIAN_POINT ( 'NONE',  ( -37.69110860217527659, -294.8896991948645336, -347.3734036179122313 ) ) ;
#37948=CARTESIAN_POINT ( 'NONE',  ( -38.67910699160877641, -288.0152243189778005, -195.7155332092584672 ) ) ;
#37950=CARTESIAN_POINT ( 'NONE',  ( 35.65787339142939771, -296.4086741954485547, -190.3901485728259217 ) ) ;
#37951=CARTESIAN_POINT ( 'NONE',  ( -112.9964973706912872, -277.3147261177873588, -282.9247227295463745 ) ) ;
#37952=ADVANCED_FACE ( 'NONE', ( #46328, #16997 ), #23164, .F. ) ;
#37953=CARTESIAN_POINT ( 'NONE',  ( -6.195093308072523008, -290.8544599722134762, -200.8032537155962132 ) ) ;
#37954=CARTESIAN_POINT ( 'NONE',  ( -77.44243007871132534, -287.0239615608816734, -208.4730675298639540 ) ) ;
#37955=CARTESIAN_POINT ( 'NONE',  ( -110.9766454386635530, -280.4159613647066180, -262.3939060166317745 ) ) ;
#37956=CARTESIAN_POINT ( 'NONE',  ( 28.18384245165263025, -288.4596801626459524, -230.9525018236989808 ) ) ;
#37957=CARTESIAN_POINT ( 'NONE',  ( 35.03716794658999589, -283.2990262911592936, -250.6575272160768577 ) ) ;
#37958=CARTESIAN_POINT ( 'NONE',  ( -2.723208958902804788, -276.7739047820277278, -339.1548632472157578 ) ) ;
#37959=CARTESIAN_POINT ( 'NONE',  ( -93.97625537493581760, -295.2494424698325588, -221.7166372947169179 ) ) ;
#37960=CARTESIAN_POINT ( 'NONE',  ( -91.05664768868534509, -279.1481685183265995, -215.1170099280971044 ) ) ;
#37961=CARTESIAN_POINT ( 'NONE',  ( -95.59315608801429676, -299.1141109904908717, -224.0137115754118042 ) ) ;
#37963=CARTESIAN_POINT ( 'NONE',  ( -69.91165696735023971, -282.1233781216988064, -202.8022627189028810 ) ) ;
#37964=CARTESIAN_POINT ( 'NONE',  ( -70.93438238202305968, -271.8548706035268197, -202.2031711506399176 ) ) ;
#37966=CARTESIAN_POINT ( 'NONE',  ( -108.8262838897055644, -277.8608066030098485, -285.4588902117479847 ) ) ;
#37967=CARTESIAN_POINT ( 'NONE',  ( -52.48223583661943792, -275.0675880126790958, -195.2151923003513616 ) ) ;
#37968=CARTESIAN_POINT ( 'NONE',  ( 37.45097726468010535, -280.3933772174981414, -253.0153047186524020 ) ) ;
#37969=CARTESIAN_POINT ( 'NONE',  ( -78.72266164990936943, -291.3777989225558827, -331.7872096583340635 ) ) ;
#37970=CARTESIAN_POINT ( 'NONE',  ( -31.98970937299928963, -299.6381229907490820, -194.0530915948497750 ) ) ;
#37971=CARTESIAN_POINT ( 'NONE',  ( -93.38279730261572809, -298.4735073980250490, -218.0591730620326985 ) ) ;
#37972=CARTESIAN_POINT ( 'NONE',  ( 26.39635497366114336, -295.0238672210218738, -231.0519721495477086 ) ) ;
#37973=CARTESIAN_POINT ( 'NONE',  ( -2.797170243721856853, -280.5943139258583869, -336.7584817938143260 ) ) ;
#37974=CARTESIAN_POINT ( 'NONE',  ( 32.41123328122457536, -283.1305321615582784, -244.2163960166066659 ) ) ;
#37975=CARTESIAN_POINT ( 'NONE',  ( -33.94107478962236968, -272.1152532615171822, -195.7938158184799420 ) ) ;
#37976=CARTESIAN_POINT ( 'NONE',  ( -98.71218438183289834, -286.7596084585323410, -225.1067590509952367 ) ) ;
#37977=CARTESIAN_POINT ( 'NONE',  ( -84.89595159269639169, -288.6462206336403256, -326.2207769746805184 ) ) ;
#37978=CARTESIAN_POINT ( 'NONE',  ( 169.3780306774251585, 231.6620261969012518, -192.5545122492718235 ) ) ;
#37980=CARTESIAN_POINT ( 'NONE',  ( -41.74488444491926487, -287.6813047203755218, -346.6580397196959780 ) ) ;
#37981=CARTESIAN_POINT ( 'NONE',  ( -0.9845994714391579361, -288.2223261237656970, -333.7458427672590915 ) ) ;
#37983=CARTESIAN_POINT ( 'NONE',  ( -21.06303720827952120, -287.3359878590978838, -195.4178218019410451 ) ) ;
#37984=CARTESIAN_POINT ( 'NONE',  ( 35.66395734434348697, -275.8656034421017011, -268.8573016045793338 ) ) ;
#37985=CARTESIAN_POINT ( 'NONE',  ( -84.06708826913678934, -290.3475395861378843, -209.4811169698811284 ) ) ;
#37986=CARTESIAN_POINT ( 'NONE',  ( 39.08050112270579746, -282.0907634891744920, -261.3536578646687758 ) ) ;
#37987=CARTESIAN_POINT ( 'NONE',  ( 19.59830107522506637, -282.3770738116945154, -219.5424215642073307 ) ) ;
#37988=CARTESIAN_POINT ( 'NONE',  ( -55.69302733148930429, -283.6154267302645167, -345.1205527136312412 ) ) ;
#37989=CARTESIAN_POINT ( 'NONE',  ( -1.966078159314026408, -280.5346557561970826, -206.5053009388257692 ) ) ;
#37990=CARTESIAN_POINT ( 'NONE',  ( -67.68488546085839630, -295.1237833571632336, -207.2794874003663779 ) ) ;
#37991=CARTESIAN_POINT ( 'NONE',  ( 202.4862527844790918, 293.5851137920426481, -83.23994149847183621 ) ) ;
#37994=CARTESIAN_POINT ( 'NONE',  ( 34.27822788303749491, -277.8330348413301749, -292.0992371250971473 ) ) ;
#37995=CARTESIAN_POINT ( 'NONE',  ( -78.78026294810004515, -207.9127932031447585, -356.5521822105918659 ) ) ;
#37996=CARTESIAN_POINT ( 'NONE',  ( -63.10763767576398209, -297.0562292587401316, -201.8969743661794496 ) ) ;
#37997=CARTESIAN_POINT ( 'NONE',  ( 39.38017149039897902, -292.9875991775623447, -264.5921216702219567 ) ) ;
#37998=CARTESIAN_POINT ( 'NONE',  ( 185.4443931024105154, 260.3151622445499243, -151.1883627937757524 ) ) ;
#37999=CARTESIAN_POINT ( 'NONE',  ( -51.67217270728417589, -296.4471537263942764, -195.2522580918571578 ) ) ;
#38000=CARTESIAN_POINT ( 'NONE',  ( -111.1372252583517053, -288.9414081907249852, -271.1740655560380446 ) ) ;
#38001=CARTESIAN_POINT ( 'NONE',  ( -107.1406086838903917, -298.0796573429769865, -295.7901449906062226 ) ) ;
#38002=CARTESIAN_POINT ( 'NONE',  ( 32.73882718537697656, -288.5753709002102028, -248.1839057564806694 ) ) ;
#38004=CARTESIAN_POINT ( 'NONE',  ( -37.67588714652610093, -295.9974518625468818, -347.1381360191537055 ) ) ;
#38005=CARTESIAN_POINT ( 'NONE',  ( -110.3710226115697708, -285.0730970311594774, -268.1916712630496704 ) ) ;
#38006=CARTESIAN_POINT ( 'NONE',  ( -99.58988748450602202, -295.9417837305581997, -225.7161642925951810 ) ) ;
#38007=CARTESIAN_POINT ( 'NONE',  ( -84.17603890807394862, -292.2297406332108949, -209.3785076887394894 ) ) ;
#38008=CARTESIAN_POINT ( 'NONE',  ( 8.808999987652043728, -293.1580491083669244, -208.7345788021393957 ) ) ;
#38009=CARTESIAN_POINT ( 'NONE',  ( -101.1247101860493416, -291.2055745553146835, -234.7505614426116551 ) ) ;
#38012=CARTESIAN_POINT ( 'NONE',  ( -105.4140822479478317, -298.8466545130112308, -237.0976805429417311 ) ) ;
#38013=CARTESIAN_POINT ( 'NONE',  ( -13.17314441254772284, -273.1542339601764411, -197.6707497586970419 ) ) ;
#38016=CARTESIAN_POINT ( 'NONE',  ( 8.199586888363507242, -275.9557434701049488, -332.4393170127128769 ) ) ;
#38017=CARTESIAN_POINT ( 'NONE',  ( -85.82050341148772077, -271.7678419455719450, -214.6491010855486934 ) ) ;
#38018=CARTESIAN_POINT ( 'NONE',  ( -106.6763083332015327, -280.7625981916240221, -243.6919817331335025 ) ) ;
#38019=CARTESIAN_POINT ( 'NONE',  ( -10.83475279343434217, -274.8423747250193969, -339.7026439493652674 ) ) ;
#38020=CARTESIAN_POINT ( 'NONE',  ( -82.19885496673704495, -298.6300005771332735, -212.2022350942222033 ) ) ;
#38021=CARTESIAN_POINT ( 'NONE',  ( -102.2445098675298283, -273.9549306473553543, -236.3243581427655045 ) ) ;
#38022=CARTESIAN_POINT ( 'NONE',  ( -26.37381662821301376, -299.7874194203834008, -194.1581838898675301 ) ) ;
#38024=CARTESIAN_POINT ( 'NONE',  ( 18.82708103143630751, -272.8754507414665227, -220.0502045523545860 ) ) ;
#38025=CARTESIAN_POINT ( 'NONE',  ( -104.0262027689579583, -296.7991953022923894, -300.4359476478604165 ) ) ;
#38026=CARTESIAN_POINT ( 'NONE',  ( -64.27046450102136532, -290.2684964245506194, -201.8623214280431455 ) ) ;
#38028=CARTESIAN_POINT ( 'NONE',  ( -20.13376311645589212, -277.3292412974519721, -345.4052188263205494 ) ) ;
#38029=CARTESIAN_POINT ( 'NONE',  ( 13.49513530746693846, -274.9551107504381093, -217.9720335527587451 ) ) ;
#38031=CARTESIAN_POINT ( 'NONE',  ( -110.6403524020426801, -282.9595852846330217, -292.3293688976641533 ) ) ;
#38032=CARTESIAN_POINT ( 'NONE',  ( -112.4014047878844167, -298.4897306950653615, -275.2462256535673077 ) ) ;
#38035=CARTESIAN_POINT ( 'NONE',  ( -46.73549448923062499, -285.1271442305770165, -197.7543325333487871 ) ) ;
#38036=CARTESIAN_POINT ( 'NONE',  ( -47.04552479385017705, -281.1749854343948982, -344.8987877324399847 ) ) ;
#38037=CARTESIAN_POINT ( 'NONE',  ( -108.0918309486891928, -276.5060405219413155, -292.2675135468204530 ) ) ;
#38038=CARTESIAN_POINT ( 'NONE',  ( -51.41117104690651729, -275.8103227967047815, -342.5928624138286409 ) ) ;
#38039=CARTESIAN_POINT ( 'NONE',  ( 12.97923336959364171, -282.7545632186796638, -214.6792131050404748 ) ) ;
#38040=CARTESIAN_POINT ( 'NONE',  ( -6.375337126376237507, -275.6733370884547298, -203.8162844600482231 ) ) ;
#38042=CARTESIAN_POINT ( 'NONE',  ( -109.3392502214157815, -271.2699654632976944, -245.4052931082674718 ) ) ;
#38043=CARTESIAN_POINT ( 'NONE',  ( -2.020010472000925983, -282.5189682774783364, -204.0104837070591657 ) ) ;
#38045=CARTESIAN_POINT ( 'NONE',  ( 28.85793303929712295, -288.9902804529170339, -233.8256666176858118 ) ) ;
#38047=CARTESIAN_POINT ( 'NONE',  ( -77.36554666504912348, -287.5883757774195715, -333.8490403940427882 ) ) ;
#38049=CARTESIAN_POINT ( 'NONE',  ( 52.29403391987453631, -297.9936773689175311, -196.9829468324793709 ) ) ;
#38050=CARTESIAN_POINT ( 'NONE',  ( -107.2028677025591747, -288.3629464893806471, -295.4665505462839974 ) ) ;
#38051=CARTESIAN_POINT ( 'NONE',  ( 197.9737475143014365, 296.4634315385704895, -68.42128063630356394 ) ) ;
#38052=CARTESIAN_POINT ( 'NONE',  ( -39.19284143790798680, -296.0287923942119050, -195.3712127120207356 ) ) ;
#38053=CARTESIAN_POINT ( 'NONE',  ( 36.11169830780685430, -286.2939863111757859, -291.0803737606623258 ) ) ;
#38054=CARTESIAN_POINT ( 'NONE',  ( -21.19353604100142974, -284.4418195411456054, -342.4253500997595552 ) ) ;
#38055=CARTESIAN_POINT ( 'NONE',  ( -60.18366881432676507, -284.0000331656657977, -197.8340883321860701 ) ) ;
#38056=CARTESIAN_POINT ( 'NONE',  ( -67.80119068360822610, -291.6409105054428892, -204.0056966741539384 ) ) ;
#38057=CARTESIAN_POINT ( 'NONE',  ( 20.97180445537994942, -282.3504855144262820, -225.4528947625408648 ) ) ;
#38058=CARTESIAN_POINT ( 'NONE',  ( 33.26674139174349421, -282.1018918807884006, -251.1546712788251909 ) ) ;
#38059=ADVANCED_FACE ( 'NONE', ( #16077, #3250 ), #31221, .F. ) ;
#38060=CARTESIAN_POINT ( 'NONE',  ( -110.6564373829958754, -292.3087541750309697, -287.8333740428198553 ) ) ;
#38061=CARTESIAN_POINT ( 'NONE',  ( -33.33661474827648163, -298.2676784322164849, -193.3610081594396206 ) ) ;
#38063=CARTESIAN_POINT ( 'NONE',  ( 26.21996961618841482, -286.1793335361921322, -311.3137351565780477 ) ) ;
#38064=CARTESIAN_POINT ( 'NONE',  ( 19.87720214335996971, -276.2517535795547019, -321.9075151797589456 ) ) ;
#38065=CARTESIAN_POINT ( 'NONE',  ( -73.44409134452433818, -293.5510314178607132, -204.9695415175167170 ) ) ;
#38067=CARTESIAN_POINT ( 'NONE',  ( -85.28047601435908120, -280.1948066931273047, -330.5268031993605859 ) ) ;
#38068=CARTESIAN_POINT ( 'NONE',  ( -72.01812765988987053, -275.5093619164914571, -337.0656063798820696 ) ) ;
#38070=CARTESIAN_POINT ( 'NONE',  ( -43.20762621294778683, -296.3792661677754836, -194.3345750951777973 ) ) ;
#38071=CARTESIAN_POINT ( 'NONE',  ( -94.68751698953826690, -272.5396184233964618, -225.0251503953136023 ) ) ;
#38072=CARTESIAN_POINT ( 'NONE',  ( -103.0363452464017939, -292.5228295113558943, -236.8576611911791190 ) ) ;
#38073=CARTESIAN_POINT ( 'NONE',  ( -104.9248197460980521, -291.8721990889911808, -242.0168600270522177 ) ) ;
#38074=CARTESIAN_POINT ( 'NONE',  ( -109.4068923262737769, -286.0921486355181287, -287.2859794326822112 ) ) ;
#38075=CARTESIAN_POINT ( 'NONE',  ( 1.385683880272469359, -293.9838099719196407, -204.4311199512791575 ) ) ;
#38076=CARTESIAN_POINT ( 'NONE',  ( 15.08794424837540582, -294.0883033630243517, -214.5709747507284817 ) ) ;
#38077=CARTESIAN_POINT ( 'NONE',  ( 35.42426483371428958, -293.4625202886259103, -276.2018668788093123 ) ) ;
#38078=CARTESIAN_POINT ( 'NONE',  ( 25.93914211147642490, -290.0940410217154408, -310.6169952348456036 ) ) ;
#38079=CARTESIAN_POINT ( 'NONE',  ( 36.59912542331345975, -281.4488246690619349, -248.8253842194818048 ) ) ;
#38080=CARTESIAN_POINT ( 'NONE',  ( -54.24873108733295624, -295.9164900576541299, -196.7169294862655420 ) ) ;
#38081=CARTESIAN_POINT ( 'NONE',  ( -78.52067087794172551, -285.3473135554751252, -205.2973617700632758 ) ) ;
#38082=CARTESIAN_POINT ( 'NONE',  ( 22.79159058339396182, -276.9260289539328710, -226.1363042096109552 ) ) ;
#38084=CARTESIAN_POINT ( 'NONE',  ( -108.4093102378187439, -283.5879308475414291, -252.0164920896237390 ) ) ;
#38085=CARTESIAN_POINT ( 'NONE',  ( 28.59199460058563247, -286.0280141179491693, -306.2152749690803262 ) ) ;
#38086=CARTESIAN_POINT ( 'NONE',  ( -113.1415284369289225, -276.7123818836934106, -268.7367008472911607 ) ) ;
#38088=AXIS2_PLACEMENT_3D ( 'NONE', #54573, #83444, #62655 ) ;
#38089=CARTESIAN_POINT ( 'NONE',  ( -68.79575240390201429, -285.1347820164560289, -204.4031666728032519 ) ) ;
#38090=AXIS2_PLACEMENT_3D ( 'NONE', #15253, #22811, #9051 ) ;
#38091=CARTESIAN_POINT ( 'NONE',  ( -11.65702282940276113, -281.5842657776760802, -198.1368346254730284 ) ) ;
#38092=CARTESIAN_POINT ( 'NONE',  ( 19.44209849457770289, -287.3153057858571060, -322.0374496882692483 ) ) ;
#38093=CARTESIAN_POINT ( 'NONE',  ( 4.406193145682850698, -296.2405483440600733, -331.4764795447555343 ) ) ;
#38094=CARTESIAN_POINT ( 'NONE',  ( -71.19691223855207340, -279.0917383025974914, -338.6272518357770309 ) ) ;
#38095=CARTESIAN_POINT ( 'NONE',  ( -56.78244293940348086, -278.6127705720674044, -344.4114615685963940 ) ) ;
#38096=CARTESIAN_POINT ( 'NONE',  ( -61.79182492101748636, -277.2121412433758678, -339.1985157613461865 ) ) ;
#38097=CARTESIAN_POINT ( 'NONE',  ( -94.15242387558603809, -299.2288517715467719, -221.6323644550944607 ) ) ;
#38098=CARTESIAN_POINT ( 'NONE',  ( 36.81639763142910482, -285.4180333055808205, -259.9514766968874255 ) ) ;
#38100=CARTESIAN_POINT ( 'NONE',  ( -110.8663202425512395, -292.4061405809321741, -250.2972950319428662 ) ) ;
#38101=CARTESIAN_POINT ( 'NONE',  ( -34.30208204216661017, -293.9333656212720598, -343.6071881580551235 ) ) ;
#38103=CARTESIAN_POINT ( 'NONE',  ( -20.84752390307642500, -294.5014145718042755, -341.5471223093775279 ) ) ;
#38104=CARTESIAN_POINT ( 'NONE',  ( -66.90902328005806510, -292.7532913219158104, -199.5990807605870430 ) ) ;
#38105=CARTESIAN_POINT ( 'NONE',  ( -89.55218366008271857, -279.9438174470339504, -219.1233851949293410 ) ) ;
#38106=CARTESIAN_POINT ( 'NONE',  ( -34.75850841673518943, -297.0041160269089460, -193.6706883115846551 ) ) ;
#38107=CARTESIAN_POINT ( 'NONE',  ( 37.72725014170847402, -288.4131013318003056, -287.0935583328578673 ) ) ;
#38108=CARTESIAN_POINT ( 'NONE',  ( 22.39142333219114178, -288.5372376295240997, -318.9379997211000273 ) ) ;
#38109=CARTESIAN_POINT ( 'NONE',  ( -5.793356887292062218, -286.8119764390199862, -204.4930250025599321 ) ) ;
#38110=CARTESIAN_POINT ( 'NONE',  ( 202.9737692553709962, 295.9636489462768054, -68.65455572930012806 ) ) ;
#38111=CARTESIAN_POINT ( 'NONE',  ( 166.2108551876890488, 232.3202090705826492, -191.5262553198002138 ) ) ;
#38112=CARTESIAN_POINT ( 'NONE',  ( 167.1921940846895893, 229.9663351943898419, -189.8569236648036451 ) ) ;
#38113=CARTESIAN_POINT ( 'NONE',  ( -91.09342159657846594, -277.0374043253031004, -320.0670094650786268 ) ) ;
#38114=CARTESIAN_POINT ( 'NONE',  ( -51.35337332025960677, -276.1558680671116690, -342.3187380588741462 ) ) ;
#38115=CARTESIAN_POINT ( 'NONE',  ( -92.15102994253193458, -272.9615447619819406, -216.3085356503619039 ) ) ;
#38116=CARTESIAN_POINT ( 'NONE',  ( -20.35789830974468018, -109.6084772789823916, -359.8065553577603737 ) ) ;
#38117=CARTESIAN_POINT ( 'NONE',  ( -110.9705065649931299, -276.9747855222266821, -291.1480642736794948 ) ) ;
#38118=CARTESIAN_POINT ( 'NONE',  ( 12.74495500033551387, -296.1252341224343354, -327.5737134146771723 ) ) ;
#38119=CARTESIAN_POINT ( 'NONE',  ( -109.6829969018154856, -290.9084358417952672, -280.6843532465209705 ) ) ;
#38120=CARTESIAN_POINT ( 'NONE',  ( -112.4448545765557412, -297.5592081711904484, -254.0615937859901408 ) ) ;
#38121=CARTESIAN_POINT ( 'NONE',  ( -101.1286437139368957, -273.7711920057724342, -227.3182133880806362 ) ) ;
#38122=CARTESIAN_POINT ( 'NONE',  ( -88.12726814782543272, -297.4840736525333114, -217.8517575210165660 ) ) ;
#38125=CARTESIAN_POINT ( 'NONE',  ( -14.99185207823118304, -278.6851731866643718, -342.5948391728875890 ) ) ;
#38126=CARTESIAN_POINT ( 'NONE',  ( 23.35050395498058862, -281.6922609910706683, -317.6685906046086529 ) ) ;
#38127=CARTESIAN_POINT ( 'NONE',  ( -87.75312529491488078, -280.4077368875006186, -217.0658230868243095 ) ) ;
#38128=CARTESIAN_POINT ( 'NONE',  ( -68.57805882759940630, -279.2171287941487208, -339.6448327876481699 ) ) ;
#38129=CARTESIAN_POINT ( 'NONE',  ( -90.68525089149083840, -271.7585826991801810, -219.4980614582265730 ) ) ;
#38131=CARTESIAN_POINT ( 'NONE',  ( -67.30822923370951116, -279.8145885708273113, -203.7817009153541221 ) ) ;
#38132=CARTESIAN_POINT ( 'NONE',  ( 20.70499276958092238, -277.0369178684688904, -320.7272392672297769 ) ) ;
#38133=CARTESIAN_POINT ( 'NONE',  ( 37.38987542344903403, -277.6337173131076952, -276.7008547578741968 ) ) ;
#38134=CARTESIAN_POINT ( 'NONE',  ( 18.46040732272641449, -274.8443577663598489, -322.5600748390428407 ) ) ;
#38137=CARTESIAN_POINT ( 'NONE',  ( 36.37035322322167019, -283.3312483454838571, -254.6489238649541278 ) ) ;
#38138=CARTESIAN_POINT ( 'NONE',  ( -57.69006915872256513, -290.9798938200905241, -200.0333399804792123 ) ) ;
#38139=CARTESIAN_POINT ( 'NONE',  ( -1.010383528823081134, -285.8701362197173808, -202.5868734572287337 ) ) ;
#38140=CARTESIAN_POINT ( 'NONE',  ( -45.77691269678831532, -281.4002506599366598, -343.9439112152375060 ) ) ;
#38141=CARTESIAN_POINT ( 'NONE',  ( -68.04663588475162328, -282.0381534561762464, -337.2384821573598970 ) ) ;
#38142=CARTESIAN_POINT ( 'NONE',  ( 21.49353193450845723, -285.0021332209296361, -224.7570647683890286 ) ) ;
#38143=CARTESIAN_POINT ( 'NONE',  ( 22.42797515750187642, -282.1653427034317474, -227.7616294682023863 ) ) ;
#38144=CARTESIAN_POINT ( 'NONE',  ( 24.96937362042031694, -22.70870612819967249, -344.9910381422254773 ) ) ;
#38146=CARTESIAN_POINT ( 'NONE',  ( -10.99793381436519546, -281.1143937487111089, -341.9185428627089891 ) ) ;
#38147=CARTESIAN_POINT ( 'NONE',  ( -5.332377254942230138, -296.6311619307271030, -338.2014921125468732 ) ) ;
#38148=CARTESIAN_POINT ( 'NONE',  ( -113.0712592572288884, -276.7051254908457167, -277.2170487885584294 ) ) ;
#38150=CARTESIAN_POINT ( 'NONE',  ( -83.06406019369541127, -278.3483213075222693, -327.4644804750734579 ) ) ;
#38151=CARTESIAN_POINT ( 'NONE',  ( -57.29440101855271905, -287.7955695959546460, -197.8369601348519495 ) ) ;
#38154=CARTESIAN_POINT ( 'NONE',  ( -104.7311097971390979, -292.9219864565461648, -236.0699337834114147 ) ) ;
#38156=CARTESIAN_POINT ( 'NONE',  ( 15.11238893981135689, -274.3122857521174751, -324.0391033689166420 ) ) ;
#38157=CARTESIAN_POINT ( 'NONE',  ( -69.29948947087444822, -288.6591707814179131, -340.2529659736412668 ) ) ;
#38158=CARTESIAN_POINT ( 'NONE',  ( 34.73549648865058970, -291.7443981673570761, -254.4495949386498808 ) ) ;
#38160=CARTESIAN_POINT ( 'NONE',  ( -109.0845264429125621, -277.4465791657704585, -254.3595933732700303 ) ) ;
#38161=CARTESIAN_POINT ( 'NONE',  ( -109.5052595901155854, -294.4651296394792439, -287.8299060026484995 ) ) ;
#38162=CARTESIAN_POINT ( 'NONE',  ( -109.6612311643044961, -291.6959195703931869, -283.4427428661520594 ) ) ;
#38165=CARTESIAN_POINT ( 'NONE',  ( 33.79805615685317122, -292.3849048071350012, -297.9626184323128655 ) ) ;
#38166=CARTESIAN_POINT ( 'NONE',  ( 17.47128430420026390, -288.4521454873818698, -220.9258929091162429 ) ) ;
#38167=CARTESIAN_POINT ( 'NONE',  ( -107.4237895048374156, -289.1705503211960604, -240.9931973861614551 ) ) ;
#38168=CARTESIAN_POINT ( 'NONE',  ( 19.10212196162155251, -288.3123591753166579, -223.1242302544103211 ) ) ;
#38169=DIRECTION ( 'NONE',  ( 0.000000000000000000, 0.000000000000000000, 1.000000000000000000 ) ) ;
#38170=CARTESIAN_POINT ( 'NONE',  ( 35.28574378847898174, -288.4711299979107366, -279.1847293194409758 ) ) ;
#38172=CARTESIAN_POINT ( 'NONE',  ( -93.41051579411129069, -297.8338025801376148, -320.7260867572086909 ) ) ;
#38174=CARTESIAN_POINT ( 'NONE',  ( 32.50912416915949876, -289.1609698821554275, -301.8074383155118312 ) ) ;
#38175=CARTESIAN_POINT ( 'NONE',  ( -40.90484585850677490, -278.0276661291882192, -195.0772881908005729 ) ) ;
#38176=CARTESIAN_POINT ( 'NONE',  ( -42.80043329190615964, -277.4525471246775510, -347.1461850449549615 ) ) ;
#38177=CARTESIAN_POINT ( 'NONE',  ( -35.33232595634194695, -279.7434158215249340, -193.3953584454684744 ) ) ;
#38178=CARTESIAN_POINT ( 'NONE',  ( -109.0462468928235324, -298.8003620417125035, -249.6173290969251468 ) ) ;
#38179=CARTESIAN_POINT ( 'NONE',  ( -27.55091640495669481, -284.1763831366105251, -196.0029227304790993 ) ) ;
#38180=CARTESIAN_POINT ( 'NONE',  ( -110.3351356391935383, -272.5060871493917602, -270.3605314645446924 ) ) ;
#38181=CARTESIAN_POINT ( 'NONE',  ( -52.04928822564251334, -278.0016273279152301, -197.5448404869050876 ) ) ;
#38182=CARTESIAN_POINT ( 'NONE',  ( -67.11153899471445072, -281.4422543931092946, -339.1997506313520603 ) ) ;
#38184=CARTESIAN_POINT ( 'NONE',  ( -37.14833585774874081, -275.5296226693956214, -346.6804828658507063 ) ) ;
#38185=CARTESIAN_POINT ( 'NONE',  ( -61.21968729243319984, -296.8878875091681948, -340.1328370557582161 ) ) ;
#38187=CARTESIAN_POINT ( 'NONE',  ( -61.14882776215457483, -282.2743603966768546, -343.3186621254529314 ) ) ;
#38188=CARTESIAN_POINT ( 'NONE',  ( -100.3628595697173864, -296.9812390932145263, -307.7670017612341553 ) ) ;
#38189=CARTESIAN_POINT ( 'NONE',  ( -34.08997682767452631, -299.4072287231633709, -193.8535555751990387 ) ) ;
#38190=CARTESIAN_POINT ( 'NONE',  ( -89.25422137235663911, -272.9630121942633423, -219.0076602137361022 ) ) ;
#38191=CARTESIAN_POINT ( 'NONE',  ( -5.207191147485279004, -294.4751929007266540, -202.5799045153537463 ) ) ;
#38192=CARTESIAN_POINT ( 'NONE',  ( 22.40648644523092159, -288.3706634549013188, -318.9529948112489137 ) ) ;
#38193=CARTESIAN_POINT ( 'NONE',  ( -85.86098415119855076, -277.4664998374685752, -212.3689101532220604 ) ) ;
#38194=CARTESIAN_POINT ( 'NONE',  ( -99.03040929027332595, -289.7721585397893591, -316.4644066337247068 ) ) ;
#38196=CARTESIAN_POINT ( 'NONE',  ( -109.8576196795451807, -289.4750679476808273, -280.6908118294176688 ) ) ;
#38197=CARTESIAN_POINT ( 'NONE',  ( -7.949881231717635721, -290.4370185403515734, -201.3462844993334500 ) ) ;
#38200=CARTESIAN_POINT ( 'NONE',  ( -82.58928494692568734, -289.1975188984123974, -327.7252575604900926 ) ) ;
#38202=CARTESIAN_POINT ( 'NONE',  ( -78.40674263858510074, -286.4550670128155616, -205.5037167377598166 ) ) ;
#38203=CARTESIAN_POINT ( 'NONE',  ( -67.68488546085839630, -291.9805209788416391, -333.4427485647536855 ) ) ;
#38204=CARTESIAN_POINT ( 'NONE',  ( 36.86602852210865677, -292.8576334676833994, -290.0088461502414248 ) ) ;
#38205=CARTESIAN_POINT ( 'NONE',  ( -61.06275791114273943, -284.6688200554312402, -343.1530184357202415 ) ) ;
#38206=CARTESIAN_POINT ( 'NONE',  ( -106.1744418274619903, -284.0601348321706610, -294.8232535178393618 ) ) ;
#38207=CARTESIAN_POINT ( 'NONE',  ( -101.2097353058410221, -273.2865370362063686, -227.2560281227328858 ) ) ;
#38208=CARTESIAN_POINT ( 'NONE',  ( 30.62454061274588213, -276.4934919209092641, -242.2662758217954035 ) ) ;
#38209=CARTESIAN_POINT ( 'NONE',  ( 20.63899226741434489, -290.9216286073296374, -223.3293401474844870 ) ) ;
#38210=CARTESIAN_POINT ( 'NONE',  ( -36.71735929268815823, -272.8550897420360002, -196.9542163663845713 ) ) ;
#38212=CARTESIAN_POINT ( 'NONE',  ( -49.37856652629597676, -155.6656457446864010, -366.7448178265262868 ) ) ;
#38213=CARTESIAN_POINT ( 'NONE',  ( -63.08333844951189917, -287.6345917927048390, -200.4585746506386954 ) ) ;
#38215=CARTESIAN_POINT ( 'NONE',  ( -98.02141753380104205, -297.0032661770089248, -317.2595657885099740 ) ) ;
#38216=CARTESIAN_POINT ( 'NONE',  ( -68.82634408111194091, -286.2783572065064845, -204.3729961819459504 ) ) ;
#38217=CARTESIAN_POINT ( 'NONE',  ( -82.41783001576253298, -276.7098571323332408, -332.4977635846553881 ) ) ;
#38218=CARTESIAN_POINT ( 'NONE',  ( 37.97243851665219694, -294.3980082376273231, -285.8882976108286584 ) ) ;
#38219=CARTESIAN_POINT ( 'NONE',  ( 21.15190270237869186, -285.0342599829427286, -222.2071574813568020 ) ) ;
#38220=CARTESIAN_POINT ( 'NONE',  ( 15.46726557943651592, -294.6629259380151780, -326.3696658334123981 ) ) ;
#38222=CARTESIAN_POINT ( 'NONE',  ( -85.94626496167029472, -291.6900750801716526, -215.7982516429003965 ) ) ;
#38223=DIRECTION ( 'NONE',  ( 1.000000000000000000, 0.000000000000000000, 0.000000000000000000 ) ) ;
#38226=CARTESIAN_POINT ( 'NONE',  ( 26.24832809208005813, -24.45034260818095007, -341.6199306127273303 ) ) ;
#38227=CARTESIAN_POINT ( 'NONE',  ( -107.2983151197432079, -286.4658101120140827, -239.7530354811208326 ) ) ;
#38228=CARTESIAN_POINT ( 'NONE',  ( -88.52914483777347243, -275.1952119285919025, -334.4957818155094174 ) ) ;
#38231=CARTESIAN_POINT ( 'NONE',  ( -73.96308360780625435, -282.4708357146256503, -333.9256661511798256 ) ) ;
#38232=CARTESIAN_POINT ( 'NONE',  ( 24.10433119332092744, -284.1330263689860089, -313.0742735949146436 ) ) ;
#38233=CARTESIAN_POINT ( 'NONE',  ( -110.7722160373275386, -273.8307757778172800, -270.3773979239509231 ) ) ;
#38234=CARTESIAN_POINT ( 'NONE',  ( -4.434163912197863766, -281.2017068078284296, -339.3370803435893777 ) ) ;
#38235=CARTESIAN_POINT ( 'NONE',  ( -40.00797838916162164, -284.0385879478847642, -195.7639480264176655 ) ) ;
#38236=CARTESIAN_POINT ( 'NONE',  ( -65.78583342212881746, -275.5444618774009200, -200.1244076857425682 ) ) ;
#38237=CARTESIAN_POINT ( 'NONE',  ( -110.2740881995150630, -297.1017357810082444, -266.0188591581253945 ) ) ;
#38238=CARTESIAN_POINT ( 'NONE',  ( 20.58185079837913989, -291.6034632902216117, -225.1068386577035199 ) ) ;
#38239=CARTESIAN_POINT ( 'NONE',  ( -111.2415884289707293, -279.4705056754106067, -249.0980209400465810 ) ) ;
#38240=CARTESIAN_POINT ( 'NONE',  ( 28.03050442123319286, -275.9940402596490685, -302.9631461159615355 ) ) ;
#38241=CARTESIAN_POINT ( 'NONE',  ( -48.94629074504154431, -298.8491627244250708, -194.4251155180126318 ) ) ;
#38242=CARTESIAN_POINT ( 'NONE',  ( -59.58852979488969481, -276.2540416485381911, -343.7543811530905487 ) ) ;
#38243=CARTESIAN_POINT ( 'NONE',  ( -31.54385115900521086, -124.1296239073781607, -364.1778657101933732 ) ) ;
#38244=CARTESIAN_POINT ( 'NONE',  ( -51.54890300056257502, -275.2335631807532081, -344.0553809397135296 ) ) ;
#38246=CARTESIAN_POINT ( 'NONE',  ( 10.84093783140056111, -295.8263448672410618, -329.7339507977677044 ) ) ;
#38250=CARTESIAN_POINT ( 'NONE',  ( -106.8297032076564363, -285.9426923828335134, -246.8430626459063433 ) ) ;
#38251=CARTESIAN_POINT ( 'NONE',  ( -41.49108591558039905, -284.8637311041416069, -346.2860497495687468 ) ) ;
#38252=CARTESIAN_POINT ( 'NONE',  ( 13.21603316624100799, -286.1300616758726960, -217.4915730602340318 ) ) ;
#38253=CARTESIAN_POINT ( 'NONE',  ( -90.03061317398214669, -277.6926388087219379, -218.6135886400298034 ) ) ;
#38254=CARTESIAN_POINT ( 'NONE',  ( -101.4562166480833270, -285.9075286045120947, -307.7802875325949685 ) ) ;
#38255=CARTESIAN_POINT ( 'NONE',  ( -65.05911048295058663, -278.1631735808554140, -202.0789613358016084 ) ) ;
#38256=CARTESIAN_POINT ( 'NONE',  ( -71.78731679912783648, -278.5983219187128839, -335.0879145805561734 ) ) ;
#38257=CARTESIAN_POINT ( 'NONE',  ( -81.11288322568364606, -273.9318433865227576, -211.7991527701329915 ) ) ;
#38258=CARTESIAN_POINT ( 'NONE',  ( 34.44030703506230395, -282.7027650657638560, -297.7746596684362430 ) ) ;
#38260=CARTESIAN_POINT ( 'NONE',  ( 17.17507782287434637, -281.2965836629814476, -215.9960167168562748 ) ) ;
#38264=CARTESIAN_POINT ( 'NONE',  ( 38.40462979923098175, -289.3913045430080047, -268.6881026303229874 ) ) ;
#38266=CARTESIAN_POINT ( 'NONE',  ( -66.87516899125938608, -296.8521327021429670, -203.4117984635471430 ) ) ;
#38267=CARTESIAN_POINT ( 'NONE',  ( -33.53610219977581153, -291.4474667964885839, -193.5572755580007822 ) ) ;
#38268=CARTESIAN_POINT ( 'NONE',  ( 31.63029556596134384, -285.6872523792127367, -244.2637082733112095 ) ) ;
#38269=CARTESIAN_POINT ( 'NONE',  ( -42.72499257243614323, -287.6959801609669398, -343.8041946979590193 ) ) ;
#38270=CARTESIAN_POINT ( 'NONE',  ( -19.81070340442436972, -290.5203253875714040, -198.4009697251290731 ) ) ;
#38271=CARTESIAN_POINT ( 'NONE',  ( -93.56912619919566509, -286.4235205853242405, -223.1847779027603735 ) ) ;
#38272=CARTESIAN_POINT ( 'NONE',  ( -107.8650874191867501, -276.2192798750934344, -296.0367544315753321 ) ) ;
#38273=CARTESIAN_POINT ( 'NONE',  ( 18.04914815115305515, -286.6742007915108275, -322.6898323005310658 ) ) ;
#38274=CARTESIAN_POINT ( 'NONE',  ( -65.15985027491844050, -287.6888408981169505, -200.6971229825820160 ) ) ;
#38275=CARTESIAN_POINT ( 'NONE',  ( -40.29290318095328161, -287.0889835324059618, -345.4826013574561898 ) ) ;
#38276=CARTESIAN_POINT ( 'NONE',  ( 22.00964024975775857, -283.0919163535518237, -313.2874522787940350 ) ) ;
#38277=CARTESIAN_POINT ( 'NONE',  ( -101.6606146046005392, -293.0735131239127895, -231.3620507675984754 ) ) ;
#38278=CARTESIAN_POINT ( 'NONE',  ( 82.13810571491718804, -300.3989273480411271, -193.5455884681284999 ) ) ;
#38280=CARTESIAN_POINT ( 'NONE',  ( -96.23956147004734873, -299.1186847680306187, -223.0287175365528753 ) ) ;
#38281=CARTESIAN_POINT ( 'NONE',  ( 29.12364956286375417, -280.3362722114337657, -239.6625714786590606 ) ) ;
#38282=CARTESIAN_POINT ( 'NONE',  ( 21.74119983320849414, -280.1858429236260690, -316.5586458956761362 ) ) ;
#38283=CARTESIAN_POINT ( 'NONE',  ( -37.69851085673302293, -294.2536496412075167, -347.2118646812024849 ) ) ;
#38284=CARTESIAN_POINT ( 'NONE',  ( -35.09704152150739276, -296.4805792807970306, -196.5617361290730969 ) ) ;
#38285=CARTESIAN_POINT ( 'NONE',  ( -39.21809448493219463, -275.1557312364776067, -344.7774693109050190 ) ) ;
#38286=CARTESIAN_POINT ( 'NONE',  ( -73.53075092266404056, -296.8583466739870005, -334.3267031128733606 ) ) ;
#38288=CARTESIAN_POINT ( 'NONE',  ( -97.33904415044567315, -271.7646587999304870, -223.0438377799489444 ) ) ;
#38289=CARTESIAN_POINT ( 'NONE',  ( -70.38771778888315112, -293.7215275353015613, -338.8001034058748928 ) ) ;
#38291=CARTESIAN_POINT ( 'NONE',  ( -14.68206905329882872, -293.7769330262451604, -200.3474333505411664 ) ) ;
#38293=CARTESIAN_POINT ( 'NONE',  ( -4.770355730253565518, -293.2952865419438808, -204.8360249310942720 ) ) ;
#38296=CARTESIAN_POINT ( 'NONE',  ( -110.6256133797539007, -282.3473357903983469, -287.9621785684037150 ) ) ;
#38297=CARTESIAN_POINT ( 'NONE',  ( 16.15913863187499899, -294.2659977360418679, -320.0266014895304920 ) ) ;
#38298=CARTESIAN_POINT ( 'NONE',  ( -55.70218118981227917, -283.2821991931421621, -345.1400771567944616 ) ) ;
#38299=CARTESIAN_POINT ( 'NONE',  ( 36.83627937149711329, -283.2889636592559555, -255.9756545566330601 ) ) ;
#38300=CARTESIAN_POINT ( 'NONE',  ( 2.733626958387584960, -286.2410543535992247, -204.6365985822053801 ) ) ;
#38301=CARTESIAN_POINT ( 'NONE',  ( -106.3849543886326074, -288.9312600485454823, -241.3636454860020422 ) ) ;
#38302=CARTESIAN_POINT ( 'NONE',  ( -85.28047601435908120, -270.9094976428775681, -210.1954327657594206 ) ) ;
#38303=CARTESIAN_POINT ( 'NONE',  ( -3.220396904966186025, -281.0896718150971196, -338.6284356751381779 ) ) ;
#38305=CARTESIAN_POINT ( 'NONE',  ( -79.57910719044741654, -284.1532785482091299, -210.1551150911958814 ) ) ;
#38306=CARTESIAN_POINT ( 'NONE',  ( -75.52177049016565036, -288.4694461545187778, -336.8725811825119649 ) ) ;
#38308=CARTESIAN_POINT ( 'NONE',  ( 18.59194129151673280, -295.8306440200837528, -318.5246364747315511 ) ) ;
#38309=CARTESIAN_POINT ( 'NONE',  ( -107.9749472046090233, -280.3507179817029851, -241.2140649768817298 ) ) ;
#38310=CARTESIAN_POINT ( 'NONE',  ( 23.54214447539355959, -292.1747373539700448, -314.7851444973658204 ) ) ;
#38311=CARTESIAN_POINT ( 'NONE',  ( -46.45488995043136526, -279.6001736171690482, -197.8597614123047492 ) ) ;
#38312=CARTESIAN_POINT ( 'NONE',  ( 35.48710783376738220, -294.0357408516879900, -295.5238188349825919 ) ) ;
#38314=CARTESIAN_POINT ( 'NONE',  ( -54.61129212475985639, -283.9117464541345726, -196.8011058332371306 ) ) ;
#38315=CARTESIAN_POINT ( 'NONE',  ( -61.73089623349540034, -279.3691083292260942, -341.3396322565309333 ) ) ;
#38316=CARTESIAN_POINT ( 'NONE',  ( 16.32342481155527381, -293.3248976544497282, -320.1954717306409179 ) ) ;
#38317=CARTESIAN_POINT ( 'NONE',  ( 94.80756045878979421, -297.7061134510668694, -195.4061741161222585 ) ) ;
#38321=CARTESIAN_POINT ( 'NONE',  ( 1.228735692626827136, -282.5494119252215910, -206.3937974810505409 ) ) ;
#38322=CARTESIAN_POINT ( 'NONE',  ( -55.82492791742164684, -294.8041295310868577, -341.0984725911246187 ) ) ;
#38324=CARTESIAN_POINT ( 'NONE',  ( -37.30987171927208834, -277.5523547857346784, -195.3611179825600175 ) ) ;
#38325=CARTESIAN_POINT ( 'NONE',  ( 25.20142870748443187, -274.1565618822819488, -225.7009995439237287 ) ) ;
#38326=CARTESIAN_POINT ( 'NONE',  ( 37.02901749127890696, -289.0939504823149377, -288.3690796320923369 ) ) ;
#38327=CARTESIAN_POINT ( 'NONE',  ( -96.76012430423257626, -290.9790014413030690, -227.8674726265915353 ) ) ;
#38328=CARTESIAN_POINT ( 'NONE',  ( -38.38291887026635152, -281.5589946963260672, -196.6626192903837307 ) ) ;
#38329=CARTESIAN_POINT ( 'NONE',  ( -62.31941323911313901, -275.3218859623015078, -200.9165050708860178 ) ) ;
#38330=ADVANCED_FACE ( 'NONE', ( #52507 ), #81383, .T. ) ;
#38331=CARTESIAN_POINT ( 'NONE',  ( -62.43033092924258654, -278.5134028308034431, -201.3314571112932185 ) ) ;
#38332=CARTESIAN_POINT ( 'NONE',  ( -99.56579800509847189, -272.9884573393094342, -224.9167645849021824 ) ) ;
#38333=CARTESIAN_POINT ( 'NONE',  ( -80.38285782364107490, -293.3845167254562512, -209.5626534471329023 ) ) ;
#38337=CARTESIAN_POINT ( 'NONE',  ( -25.19573484224367022, -290.3450152465179031, -195.5762197373435924 ) ) ;
#38338=CARTESIAN_POINT ( 'NONE',  ( -108.5935202911870476, -272.2728100420393389, -254.2004693157816746 ) ) ;
#38340=CARTESIAN_POINT ( 'NONE',  ( -112.1841381722990150, -291.8836891193671477, -285.3039995540744371 ) ) ;
#38341=CARTESIAN_POINT ( 'NONE',  ( -111.2869819898779866, -293.4805209788416391, -234.7871824221999191 ) ) ;
#38342=CARTESIAN_POINT ( 'NONE',  ( -41.44838100212109566, -288.0005051074205085, -195.6277357957662559 ) ) ;
#38343=CARTESIAN_POINT ( 'NONE',  ( 37.17738074211008126, -273.6401488022884223, -277.2120311342031300 ) ) ;
#38344=CARTESIAN_POINT ( 'NONE',  ( 24.98609461861684977, -276.9191967559033856, -229.6602555895457272 ) ) ;
#38345=CARTESIAN_POINT ( 'NONE',  ( 23.78408674541283219, -291.0510818093234207, -227.8539174325783847 ) ) ;
#38346=CARTESIAN_POINT ( 'NONE',  ( -8.036980334142889149, -282.2923350966429439, -200.4790360668626192 ) ) ;
#38348=CARTESIAN_POINT ( 'NONE',  ( 5.645347047554210462, -281.8007761876296513, -329.4881544632503960 ) ) ;
#38349=CARTESIAN_POINT ( 'NONE',  ( -99.39153700770440025, -279.0311643601683045, -315.4535023684555881 ) ) ;
#38350=CARTESIAN_POINT ( 'NONE',  ( 24.77625827103772238, -280.9447965455061649, -315.2093527251433898 ) ) ;
#38351=CARTESIAN_POINT ( 'NONE',  ( -70.18942206231223224, -278.4156382876280418, -339.7574056422278090 ) ) ;
#38353=CARTESIAN_POINT ( 'NONE',  ( 38.62509353769181075, -276.9747198964386712, -262.6311570143912490 ) ) ;
#38354=CARTESIAN_POINT ( 'NONE',  ( -102.0455923789670294, -293.4805209788416391, -239.2376011013261916 ) ) ;
#38356=CARTESIAN_POINT ( 'NONE',  ( -110.4316933438511370, -298.7682539757504969, -253.5428676159656050 ) ) ;
#38358=CARTESIAN_POINT ( 'NONE',  ( -110.4296494165745202, -291.5489539411085502, -276.6701365953661593 ) ) ;
#38359=CARTESIAN_POINT ( 'NONE',  ( -15.93270950355617543, -274.7941352625059608, -341.9240697206458890 ) ) ;
#38360=CARTESIAN_POINT ( 'NONE',  ( 2.665923041233587476, -290.2839707296153620, -335.0244330072943058 ) ) ;
#38361=CARTESIAN_POINT ( 'NONE',  ( -102.4966600036601960, -290.3516437447562453, -237.1020852761221249 ) ) ;
#38362=CARTESIAN_POINT ( 'NONE',  ( 37.44311689830367129, -287.2867217584202990, -288.4932048968876188 ) ) ;
#38364=CARTESIAN_POINT ( 'NONE',  ( -85.39797985797937940, -282.1294617860167477, -326.3703528610641911 ) ) ;
#38365=CARTESIAN_POINT ( 'NONE',  ( -85.46809442110621546, -291.5858348596074734, -326.9507650845525859 ) ) ;
#38366=CARTESIAN_POINT ( 'NONE',  ( -54.90297507577628267, -284.3022733159571658, -198.7380159556053059 ) ) ;
#38367=CARTESIAN_POINT ( 'NONE',  ( 7.429577419464150623, -281.9921778690282395, -212.0148708629042460 ) ) ;
#38368=CARTESIAN_POINT ( 'NONE',  ( 37.48756817190958657, -288.2778622312388279, -253.1738733812769055 ) ) ;
#38370=CARTESIAN_POINT ( 'NONE',  ( -98.04823361276523030, -279.6097408603251324, -229.6177955603075134 ) ) ;
#38371=CARTESIAN_POINT ( 'NONE',  ( -22.25688375772180194, -291.0360023838061920, -195.2040939807425843 ) ) ;
#38372=CARTESIAN_POINT ( 'NONE',  ( 38.93157505034587018, -288.4769434130623154, -280.0925696633081543 ) ) ;
#38373=CARTESIAN_POINT ( 'NONE',  ( 18.60437654828044174, -288.7663387799738075, -323.1774356101923331 ) ) ;
#38374=CARTESIAN_POINT ( 'NONE',  ( -100.4000645825083211, -284.2140654984655725, -307.1394088186335694 ) ) ;
#38377=CARTESIAN_POINT ( 'NONE',  ( -1.410869199410667685, -294.3838741617315122, -203.6581879796983401 ) ) ;
#38379=CARTESIAN_POINT ( 'NONE',  ( 27.67792636295152775, -292.7688439279630188, -310.7811613359442049 ) ) ;
#38380=AXIS2_PLACEMENT_3D ( 'NONE', #22524, #87377, #51396 ) ;
#38381=CARTESIAN_POINT ( 'NONE',  ( 26.96765282657602825, -275.0889275876850775, -305.5058730060741254 ) ) ;
#38382=CARTESIAN_POINT ( 'NONE',  ( -31.91013715723157418, -297.4670732795708545, -193.4636322180529646 ) ) ;
#38383=CARTESIAN_POINT ( 'NONE',  ( 34.44647330940923524, -292.2502373729911369, -287.0649462891273060 ) ) ;
#38384=CARTESIAN_POINT ( 'NONE',  ( -108.8083567849265023, -295.0433392946682716, -251.0641941214466613 ) ) ;
#38385=CARTESIAN_POINT ( 'NONE',  ( -106.9527213638054093, -292.0645909574458301, -247.0923357363581090 ) ) ;
#38386=CARTESIAN_POINT ( 'NONE',  ( 35.60144556126719095, -294.5292928190697808, -262.5553946875014617 ) ) ;
#38387=CARTESIAN_POINT ( 'NONE',  ( 133.0872704186301405, -299.5541904835127980, -195.3611179825600175 ) ) ;
#38389=CARTESIAN_POINT ( 'NONE',  ( -47.41178340180002948, -293.1796984736866420, -344.8501899837609699 ) ) ;
#38390=CARTESIAN_POINT ( 'NONE',  ( -66.75749003150183114, -299.6669560479044208, -201.3566650642730167 ) ) ;
#38391=CARTESIAN_POINT ( 'NONE',  ( -8.113602617729419819, -289.6010680811129987, -337.5653682545494689 ) ) ;
#38394=CARTESIAN_POINT ( 'NONE',  ( 7.287660961615398669, -278.4275849709833324, -331.1433368424354740 ) ) ;
#38395=CARTESIAN_POINT ( 'NONE',  ( -39.96480596265028140, -275.8793195343735647, -346.9321209962316175 ) ) ;
#38397=CARTESIAN_POINT ( 'NONE',  ( -49.69467705304472815, -273.2472898199230826, -194.4079987789754966 ) ) ;
#38398=CARTESIAN_POINT ( 'NONE',  ( 16.85786742071456601, -280.3531236580254813, -321.4621273476014380 ) ) ;
#38399=CARTESIAN_POINT ( 'NONE',  ( -53.97666152125205485, -275.6619971649533909, -344.7772703764786115 ) ) ;
#38400=CARTESIAN_POINT ( 'NONE',  ( -108.3075101263664806, -295.4882345872784981, -251.2051467548723167 ) ) ;
#38401=CARTESIAN_POINT ( 'NONE',  ( -95.59627442016343934, -275.2030350989207932, -223.1034399805188855 ) ) ;
#38402=CARTESIAN_POINT ( 'NONE',  ( -48.89972073598492130, -274.5525847951537344, -198.1274311562501964 ) ) ;
#38404=CARTESIAN_POINT ( 'NONE',  ( -109.6466878092473110, -288.8442713887507125, -249.1385931478510827 ) ) ;
#38405=CARTESIAN_POINT ( 'NONE',  ( 22.28205928802048774, -274.7973126082226827, -228.2205122141655522 ) ) ;
#38406=CARTESIAN_POINT ( 'NONE',  ( 25.85170750003431550, -288.1345815258399625, -314.4480433355608398 ) ) ;
#38407=CARTESIAN_POINT ( 'NONE',  ( 51.15003443965340324, -301.1346102307301749, -194.9762188656702335 ) ) ;
#38408=CARTESIAN_POINT ( 'NONE',  ( -95.01048168695832885, -295.2117324032735155, -222.6511494115316054 ) ) ;
#38409=CARTESIAN_POINT ( 'NONE',  ( -74.20751820094648110, -282.7261465352300434, -337.8376250146515645 ) ) ;
#38411=CARTESIAN_POINT ( 'NONE',  ( 37.70396000512317869, -279.5638603164040319, -271.2858296272250982 ) ) ;
#38413=CARTESIAN_POINT ( 'NONE',  ( -77.45942791351100709, -290.2954812061835241, -208.8981338247106692 ) ) ;
#38414=CARTESIAN_POINT ( 'NONE',  ( -29.33457778158224727, -281.0893635188935491, -344.2145858785827954 ) ) ;
#38417=CARTESIAN_POINT ( 'NONE',  ( -63.47437060616803706, -289.7114337277214418, -200.0611593613644743 ) ) ;
#38418=CARTESIAN_POINT ( 'NONE',  ( -36.74976385216874064, -275.5798458440512491, -196.6576269246798176 ) ) ;
#38419=CARTESIAN_POINT ( 'NONE',  ( -97.72191922565930611, -285.1240637988797744, -317.5017359469233043 ) ) ;
#38420=CARTESIAN_POINT ( 'NONE',  ( 0.4959079117829636729, -272.6320497298677878, -204.9425260007590452 ) ) ;
#38421=CARTESIAN_POINT ( 'NONE',  ( -42.67412919225751722, -285.9830368293920060, -197.5435117709969575 ) ) ;
#38422=CARTESIAN_POINT ( 'NONE',  ( 16.03768453958602436, -277.7017458304090383, -321.0169785486190790 ) ) ;
#38423=CARTESIAN_POINT ( 'NONE',  ( -8.665984192381040785, -277.4698995446594836, -337.6822321636994388 ) ) ;
#38424=CARTESIAN_POINT ( 'NONE',  ( -2.538993479511827189, -284.5919402284860666, -336.7973450088994127 ) ) ;
#38427=CARTESIAN_POINT ( 'NONE',  ( 114.7448031289451222, -299.5541904835127980, -193.0244903219134756 ) ) ;
#38428=CARTESIAN_POINT ( 'NONE',  ( -44.79773735905121157, -294.9772411305903574, -347.0526843203343219 ) ) ;
#38429=CARTESIAN_POINT ( 'NONE',  ( -49.71853397641705641, -287.8735649070609384, -196.6969030181209632 ) ) ;
#38431=CARTESIAN_POINT ( 'NONE',  ( 40.64545035920995986, -285.2666405000203440, -288.1938231032136741 ) ) ;
#38432=CARTESIAN_POINT ( 'NONE',  ( -112.6898927689198757, -277.6527757842909523, -256.0031111151678260 ) ) ;
#38433=CARTESIAN_POINT ( 'NONE',  ( -94.10165198749720616, -289.6489474031497480, -219.5206982253849333 ) ) ;
#38435=CARTESIAN_POINT ( 'NONE',  ( -101.6053319760717670, -286.5623667823225560, -234.1885920237355379 ) ) ;
#38436=CARTESIAN_POINT ( 'NONE',  ( -71.42802845166538361, -281.3557639055264872, -204.6498298136843630 ) ) ;
#38437=CARTESIAN_POINT ( 'NONE',  ( -64.35598605796496940, -287.1317016380446603, -198.8709448788910095 ) ) ;
#38438=CARTESIAN_POINT ( 'NONE',  ( 15.34737533745692240, -284.3084113693651602, -323.8089971205864686 ) ) ;
#38439=CARTESIAN_POINT ( 'NONE',  ( 33.02062984517930033, -276.1180004560837915, -301.6363881687481694 ) ) ;
#38440=CARTESIAN_POINT ( 'NONE',  ( -112.1740853773269038, -270.5882458020582817, -267.5434424033534810 ) ) ;
#38441=CARTESIAN_POINT ( 'NONE',  ( -50.93754487765809813, -279.7163340108675129, -194.5709272582197116 ) ) ;
#38443=CARTESIAN_POINT ( 'NONE',  ( -92.93631029256951592, -299.1664390810638565, -220.8580522193773277 ) ) ;
#38447=CARTESIAN_POINT ( 'NONE',  ( -112.8531441054083047, -270.8995448367077756, -261.8760816757083489 ) ) ;
#38449=CARTESIAN_POINT ( 'NONE',  ( -94.50510170511438446, -277.4175670830590548, -315.8820263994580273 ) ) ;
#38451=CARTESIAN_POINT ( 'NONE',  ( -81.03655275476577913, -274.6785734826400471, -207.3780857020441601 ) ) ;
#38452=CARTESIAN_POINT ( 'NONE',  ( 1.963337758915105979, -281.5982888175031462, -336.2999851971397334 ) ) ;
#38453=CARTESIAN_POINT ( 'NONE',  ( -45.45152568235523205, -290.9164612216891896, -343.9288061492744077 ) ) ;
#38454=CARTESIAN_POINT ( 'NONE',  ( -74.25384824107425175, -297.0533710928539222, -337.2050230729130931 ) ) ;
#38455=CARTESIAN_POINT ( 'NONE',  ( -79.24685402941869938, -296.8093402388691402, -334.4857372358493990 ) ) ;
#38456=CARTESIAN_POINT ( 'NONE',  ( 24.85108799284440195, -294.9884647037296759, -228.7427862960367122 ) ) ;
#38457=CARTESIAN_POINT ( 'NONE',  ( 30.97806932586036055, -279.9546092500733607, -301.0240919962785142 ) ) ;
#38458=CARTESIAN_POINT ( 'NONE',  ( -27.38959879430306188, -282.0996023331566676, -196.5371774006363239 ) ) ;
#38459=CARTESIAN_POINT ( 'NONE',  ( -96.41722003954978959, -295.2571237522643059, -225.0480045448180704 ) ) ;
#38460=CARTESIAN_POINT ( 'NONE',  ( -107.4826924242310753, -285.7677275432773740, -300.2732173316468334 ) ) ;
#38463=CARTESIAN_POINT ( 'NONE',  ( 19.74557775531378923, -287.1200090360013633, -316.3531692368167114 ) ) ;
#38464=CARTESIAN_POINT ( 'NONE',  ( 140.6514286645508207, 179.2331402481280236, -240.9484025443371706 ) ) ;
#38466=CARTESIAN_POINT ( 'NONE',  ( -5.885770650012288385, -287.2213916663812370, -339.9968185629729192 ) ) ;
#38467=CARTESIAN_POINT ( 'NONE',  ( 35.65093069525761393, -287.2637592726157436, -273.7650458607844826 ) ) ;
#38469=CARTESIAN_POINT ( 'NONE',  ( -102.6476277784160231, -285.1041721060128680, -310.5684347669297267 ) ) ;
#38470=CARTESIAN_POINT ( 'NONE',  ( 35.12761081617328074, -276.0089223663409825, -279.7248369698144188 ) ) ;
#38471=CARTESIAN_POINT ( 'NONE',  ( -92.57985671707740494, -290.2044330025888712, -217.0855957570606449 ) ) ;
#38472=CARTESIAN_POINT ( 'NONE',  ( 17.75903708443733464, -282.9406334571459070, -324.0769510528670594 ) ) ;
#38473=CARTESIAN_POINT ( 'NONE',  ( 1.008615363151603272, -282.0739696739936448, -204.3315720239004349 ) ) ;
#38474=CARTESIAN_POINT ( 'NONE',  ( 36.45962783886409397, -282.1621962055115205, -292.4330717640871171 ) ) ;
#38475=CARTESIAN_POINT ( 'NONE',  ( 11.30582025366161858, -280.7490792086498459, -215.9330116338370260 ) ) ;
#38476=CARTESIAN_POINT ( 'NONE',  ( -21.39648532958014826, -292.3380690714489560, -340.3683826091709079 ) ) ;
#38477=CARTESIAN_POINT ( 'NONE',  ( -77.50303971134606229, -208.8530697131320153, -357.3053013794460639 ) ) ;
#38479=CARTESIAN_POINT ( 'NONE',  ( 31.86072791008295013, -277.1783681167906366, -241.7461843042033820 ) ) ;
#38480=CARTESIAN_POINT ( 'NONE',  ( -108.3143740274736757, -261.7878351234190859, -317.3776606196656189 ) ) ;
#38481=CARTESIAN_POINT ( 'NONE',  ( 36.32278028721702867, -279.7278161541131567, -282.4189423701175770 ) ) ;
#38482=CARTESIAN_POINT ( 'NONE',  ( -107.5549654667471060, -296.1694816034614632, -250.0143728171061923 ) ) ;
#38483=CARTESIAN_POINT ( 'NONE',  ( 21.31666403547346178, -293.7314648761540639, -320.1478955151795844 ) ) ;
#38484=CARTESIAN_POINT ( 'NONE',  ( 154.1818069414172783, 204.3837156544556422, -214.5532738587077404 ) ) ;
#38485=CARTESIAN_POINT ( 'NONE',  ( -34.06005215504181649, -296.6672129428951052, -193.9511196260665145 ) ) ;
#38486=CARTESIAN_POINT ( 'NONE',  ( -91.19028885873797208, -288.2330510603243852, -320.9013010507957233 ) ) ;
#38487=CARTESIAN_POINT ( 'NONE',  ( -0.1184100674215761706, -296.4121496192478276, -334.6482339227985108 ) ) ;
#38488=CARTESIAN_POINT ( 'NONE',  ( 11.44902650208045181, -288.0604527573427163, -215.3317840669182317 ) ) ;
#38491=CARTESIAN_POINT ( 'NONE',  ( 38.61728129580925639, -294.3497738350770874, -258.9118917159863145 ) ) ;
#38492=CARTESIAN_POINT ( 'NONE',  ( -69.03018709037934286, -283.9728641881617364, -336.2067496658171990 ) ) ;
#38493=CARTESIAN_POINT ( 'NONE',  ( -57.27154210512010479, -296.5955917733255092, -196.3412025614190100 ) ) ;
#38494=CARTESIAN_POINT ( 'NONE',  ( 4.045928813690177428, -293.3970060694782660, -205.5583997515548162 ) ) ;
#38495=CARTESIAN_POINT ( 'NONE',  ( 38.26360101978755068, -293.8660056368633491, -256.1004959158440784 ) ) ;
#38496=CARTESIAN_POINT ( 'NONE',  ( -69.97054427848298985, -289.6610254597630387, -335.6770329349184863 ) ) ;
#38497=VERTEX_POINT ( 'NONE', #19795 ) ;
#38499=CARTESIAN_POINT ( 'NONE',  ( -67.70457009757159028, -299.5185176082915746, -200.8905144143280097 ) ) ;
#38500=CARTESIAN_POINT ( 'NONE',  ( -73.74257889085031081, -272.3752130129523152, -202.9004891753010895 ) ) ;
#38501=CARTESIAN_POINT ( 'NONE',  ( 18.66658292093065796, -281.2792539473255147, -317.5661790417046859 ) ) ;
#38504=CARTESIAN_POINT ( 'NONE',  ( -42.80805925910741649, -276.6270520138905340, -347.1051459007585436 ) ) ;
#38505=CARTESIAN_POINT ( 'NONE',  ( -40.79216921455333278, -272.4080364295741674, -196.5915752667416427 ) ) ;
#38506=CARTESIAN_POINT ( 'NONE',  ( -62.75367302011007808, -281.5784002811615210, -200.5566020078079248 ) ) ;
#38507=CARTESIAN_POINT ( 'NONE',  ( -69.81273757450152573, -275.6238710964494771, -337.1321920999869803 ) ) ;
#38508=CARTESIAN_POINT ( 'NONE',  ( -94.77155617724071135, -298.3991484513010732, -224.6561714183339689 ) ) ;
#38509=CARTESIAN_POINT ( 'NONE',  ( -21.89605366827960964, -275.1962368745994354, -198.7731270007397484 ) ) ;
#38510=CARTESIAN_POINT ( 'NONE',  ( -112.5447892850460505, -274.4547872134068029, -259.1171465317853517 ) ) ;
#38511=CARTESIAN_POINT ( 'NONE',  ( -35.53734438785662775, -272.0947688877483870, -195.0146697697466038 ) ) ;
#38512=CARTESIAN_POINT ( 'NONE',  ( 27.57325502563815789, -293.7470686021507049, -236.7465189929239386 ) ) ;
#38513=CARTESIAN_POINT ( 'NONE',  ( 34.52917583849760774, -291.9192259512259966, -254.4929129107979975 ) ) ;
#38514=CARTESIAN_POINT ( 'NONE',  ( -6.593530494673972342, -277.1514734525161998, -340.9024997457509585 ) ) ;
#38516=CARTESIAN_POINT ( 'NONE',  ( 34.84133724452625103, -275.5740562193524852, -259.3862464096388862 ) ) ;
#38517=CARTESIAN_POINT ( 'NONE',  ( -93.08378595305521230, -282.5169859453421282, -322.7837460224268966 ) ) ;
#38518=CARTESIAN_POINT ( 'NONE',  ( 37.67440604498001022, -295.6230021717669274, -275.8785845459177040 ) ) ;
#38520=CARTESIAN_POINT ( 'NONE',  ( -38.61749165448306087, -285.2329497985221565, -197.1982559707703899 ) ) ;
#38522=CARTESIAN_POINT ( 'NONE',  ( -98.31659834280573307, -281.9539909832136004, -314.4036871802330211 ) ) ;
#38523=CARTESIAN_POINT ( 'NONE',  ( 31.80927144240720850, -274.4613172570902293, -295.6788772234957037 ) ) ;
#38524=CARTESIAN_POINT ( 'NONE',  ( 26.04886463930497698, -284.0925361584082793, -310.5397254766070319 ) ) ;
#38525=CARTESIAN_POINT ( 'NONE',  ( 33.23761890483539361, -276.4902060105467285, -250.0378959275174680 ) ) ;
#38528=CARTESIAN_POINT ( 'NONE',  ( -67.20316549286576446, -272.0669709513870771, -200.2559590933015841 ) ) ;
#38530=CARTESIAN_POINT ( 'NONE',  ( -110.0474838609024602, -280.3071135841789214, -289.4877220180256359 ) ) ;
#38532=CARTESIAN_POINT ( 'NONE',  ( -24.06344875422471219, -288.1404764920047796, -195.9237649757746738 ) ) ;
#38533=CARTESIAN_POINT ( 'NONE',  ( -91.68632222370136731, -289.2779664695461861, -218.5995970954718359 ) ) ;
#38536=CARTESIAN_POINT ( 'NONE',  ( -110.7816523572172400, -295.3327331340378805, -271.4537965941055404 ) ) ;
#38537=CARTESIAN_POINT ( 'NONE',  ( 14.93672385205651310, -286.4449433155193105, -323.0662587696817809 ) ) ;
#38538=CARTESIAN_POINT ( 'NONE',  ( 81.08292338999881110, 82.25620239566015357, -296.3357184930298445 ) ) ;
#38539=CARTESIAN_POINT ( 'NONE',  ( -53.02922665931427559, -295.8510235811711482, -196.9668153148425915 ) ) ;
#38540=CARTESIAN_POINT ( 'NONE',  ( 36.82590184792485388, -286.2591133026817829, -288.3571208871751992 ) ) ;
#38541=CARTESIAN_POINT ( 'NONE',  ( -0.8387789176852811224, -284.1588570990017502, -334.5014107697758732 ) ) ;
#38542=CARTESIAN_POINT ( 'NONE',  ( -24.72420871733400105, -281.1332925138557357, -345.3463077315985288 ) ) ;
#38543=CARTESIAN_POINT ( 'NONE',  ( -110.2456556156483174, -290.6131701911235723, -265.7356183765746209 ) ) ;
#38544=CARTESIAN_POINT ( 'NONE',  ( 28.68772571341341404, -283.4155053428108317, -302.9651208116308112 ) ) ;
#38545=CARTESIAN_POINT ( 'NONE',  ( 22.72317268907492505, -282.9358917705762906, -312.1320741675502859 ) ) ;
#38546=CARTESIAN_POINT ( 'NONE',  ( -96.84496032399584919, -291.9010471635554040, -316.5971302783976284 ) ) ;
#38547=CARTESIAN_POINT ( 'NONE',  ( 76.38462255090273345, -299.6058777463841807, -193.3579203087136023 ) ) ;
#38548=CARTESIAN_POINT ( 'NONE',  ( -0.01378055072520428456, -286.6397010727742440, -336.1160537688457453 ) ) ;
#38549=CARTESIAN_POINT ( 'NONE',  ( 1.195421383891718481, -274.5518939205146012, -203.6833226859605759 ) ) ;
#38550=CARTESIAN_POINT ( 'NONE',  ( -14.36349944652816113, -294.3314635687355576, -199.3410567722573887 ) ) ;
#38552=CARTESIAN_POINT ( 'NONE',  ( -110.4542110544635705, -286.8376638359844719, -287.0812184334320705 ) ) ;
#38553=CARTESIAN_POINT ( 'NONE',  ( -35.77586197230581178, -275.0324271114433259, -345.5242892143131712 ) ) ;
#38555=CARTESIAN_POINT ( 'NONE',  ( -94.95274135883745714, -295.6335435708235195, -220.4084700009051403 ) ) ;
#38556=CARTESIAN_POINT ( 'NONE',  ( -111.1686156865934691, -292.1770787729165022, -268.4612761058797332 ) ) ;
#38557=CARTESIAN_POINT ( 'NONE',  ( -56.88089049190765678, -273.1421516632114503, -199.8660645403049898 ) ) ;
#38558=CARTESIAN_POINT ( 'NONE',  ( -109.1070615161358006, -292.2918290585453747, -253.5596638670428149 ) ) ;
#38559=CARTESIAN_POINT ( 'NONE',  ( -12.19062214125767696, -293.3287104482897689, -201.5260284210976920 ) ) ;
#38560=CARTESIAN_POINT ( 'NONE',  ( -94.18614826009915930, -285.6488851040086274, -317.7603029178505949 ) ) ;
#38561=CARTESIAN_POINT ( 'NONE',  ( -68.10829382968361756, -293.0812967459226002, -200.4038609825165054 ) ) ;
#38562=CARTESIAN_POINT ( 'NONE',  ( -92.46844943382534154, -292.5988922430018988, -217.2353785349184818 ) ) ;
#38563=CARTESIAN_POINT ( 'NONE',  ( -36.99768062687767411, -294.8810132462169804, -343.3727315176086563 ) ) ;
#38564=CARTESIAN_POINT ( 'NONE',  ( 22.79190936736363682, -290.1646338507283076, -315.2039335150693660 ) ) ;
#38565=CARTESIAN_POINT ( 'NONE',  ( 37.19234088328034460, -281.9607734364608973, -289.6918379650740007 ) ) ;
#38566=CARTESIAN_POINT ( 'NONE',  ( -88.61290497509071429, -295.4198626974820172, -214.7873107050126862 ) ) ;
#38567=CARTESIAN_POINT ( 'NONE',  ( -112.9978370375786199, -284.5680260334411855, -255.7607145945312084 ) ) ;
#38568=CARTESIAN_POINT ( 'NONE',  ( 22.16304058319692061, -278.1513666033033019, -315.4280974550524093 ) ) ;
#38569=CARTESIAN_POINT ( 'NONE',  ( -110.2690933549070849, -283.2325396760733724, -279.0904278785691304 ) ) ;
#38570=CARTESIAN_POINT ( 'NONE',  ( 16.92253023958250679, -284.8245188364819569, -218.5136701463097211 ) ) ;
#38571=CARTESIAN_POINT ( 'NONE',  ( -111.2841899529980481, -276.4818060341775094, -286.8781904642541463 ) ) ;
#38572=CARTESIAN_POINT ( 'NONE',  ( -7.233842321018532751, -282.1539144287816043, -336.9443951218236748 ) ) ;
#38573=CARTESIAN_POINT ( 'NONE',  ( -107.0641171735762782, -280.1663306701457259, -238.5033434644013255 ) ) ;
#38574=CARTESIAN_POINT ( 'NONE',  ( 23.94709541931997521, -287.2283074292884635, -316.5834475868662139 ) ) ;
#38575=CARTESIAN_POINT ( 'NONE',  ( 29.31681280234223408, -295.7430141291494010, -302.6448433069928683 ) ) ;
#38576=CARTESIAN_POINT ( 'NONE',  ( -45.54304751212969649, -278.7544228478503214, -346.1709895120840201 ) ) ;
#38577=CARTESIAN_POINT ( 'NONE',  ( -2.795305985376551838, -275.8143117622976206, -202.0834538698937877 ) ) ;
#38578=CARTESIAN_POINT ( 'NONE',  ( -110.3511100643348186, -278.4178561801667229, -267.9061455862392336 ) ) ;
#38579=CARTESIAN_POINT ( 'NONE',  ( -100.6893832978647367, -275.0649569870145683, -230.8779843866845738 ) ) ;
#38580=CARTESIAN_POINT ( 'NONE',  ( 36.32199364678888998, -285.7215866698029458, -283.5402168862246981 ) ) ;
#38581=CARTESIAN_POINT ( 'NONE',  ( -112.1435947867584275, -292.3367591503438234, -255.7631879635000587 ) ) ;
#38582=CARTESIAN_POINT ( 'NONE',  ( 26.05310986494746572, -292.9754349837666609, -307.1758451841873807 ) ) ;
#38584=CARTESIAN_POINT ( 'NONE',  ( 34.23805766763726410, -293.0284775758734099, -255.9241598278603078 ) ) ;
#38586=CARTESIAN_POINT ( 'NONE',  ( -51.61424574545161903, -290.3102894950367272, -345.7122092189596856 ) ) ;
#38587=CARTESIAN_POINT ( 'NONE',  ( -43.76830648553805503, -280.6203495924389699, -197.4919193750880595 ) ) ;
#38588=CARTESIAN_POINT ( 'NONE',  ( -82.77634124440942287, -296.3678004105220225, -208.5117659198416220 ) ) ;
#38589=CARTESIAN_POINT ( 'NONE',  ( 38.45497851479283469, -288.0401919739044843, -257.3154214071294064 ) ) ;
#38590=CARTESIAN_POINT ( 'NONE',  ( -57.28132837293846080, -289.6357799515886313, -344.7677740555731134 ) ) ;
#38591=CARTESIAN_POINT ( 'NONE',  ( -66.56413762178077320, -283.7790208351960928, -337.2935735189538491 ) ) ;
#38592=CARTESIAN_POINT ( 'NONE',  ( -40.04897441875193209, -139.4172891677515622, -364.6093070308701272 ) ) ;
#38593=CARTESIAN_POINT ( 'NONE',  ( -104.9560684206034011, -254.4573753784908376, -325.6091621043333362 ) ) ;
#38594=CARTESIAN_POINT ( 'NONE',  ( -83.13117446773537722, -218.5196643677905968, -348.8949988116463032 ) ) ;
#38595=CARTESIAN_POINT ( 'NONE',  ( -35.12295939574989490, -276.2207464307940654, -343.4889438559031873 ) ) ;
#38596=CARTESIAN_POINT ( 'NONE',  ( -107.9121576436898380, -277.7343136329654953, -250.4642683499850193 ) ) ;
#38597=CARTESIAN_POINT ( 'NONE',  ( -20.52033662665390423, -297.7651257057431735, -193.4240162007132824 ) ) ;
#38598=CARTESIAN_POINT ( 'NONE',  ( 190.4953182115862376, 268.1230253924587146, -138.0059063792686516 ) ) ;
#38599=CARTESIAN_POINT ( 'NONE',  ( -31.50471103718881949, -275.6648754719511203, -346.6972678698147661 ) ) ;
#38601=CARTESIAN_POINT ( 'NONE',  ( -107.7834588917727956, -290.7863070775582059, -289.9368497607976565 ) ) ;
#38602=CARTESIAN_POINT ( 'NONE',  ( -35.84235262091186769, -298.8733041410477540, -193.5223946047195227 ) ) ;
#38603=CARTESIAN_POINT ( 'NONE',  ( 35.44647769315002250, -286.3712344419290616, -280.6076267911944342 ) ) ;
#38604=CARTESIAN_POINT ( 'NONE',  ( -110.9419918742206761, -273.4856394004074787, -247.9010192517368978 ) ) ;
#38605=CARTESIAN_POINT ( 'NONE',  ( -63.56701120472439470, -295.5702629216104356, -338.5412712193190714 ) ) ;
#38608=CARTESIAN_POINT ( 'NONE',  ( -68.40068826831367232, -279.3771157487001915, -339.2566956689610720 ) ) ;
#38610=CARTESIAN_POINT ( 'NONE',  ( -27.38628060855530322, -282.4366715455404915, -346.7060905660006824 ) ) ;
#38611=CARTESIAN_POINT ( 'NONE',  ( -105.5503977577082253, -279.2740471069772639, -297.2274471070107893 ) ) ;
#38612=CARTESIAN_POINT ( 'NONE',  ( -111.7302058166181524, -280.5095439326133260, -254.7958839262545325 ) ) ;
#38613=CARTESIAN_POINT ( 'NONE',  ( -110.5726122726317584, -271.1397352805959144, -262.1184692380630850 ) ) ;
#38614=CARTESIAN_POINT ( 'NONE',  ( 18.83474343374798821, -281.0574907321378078, -223.7240476879092910 ) ) ;
#38615=CARTESIAN_POINT ( 'NONE',  ( -60.83150259239849333, -274.5578704625709179, -197.1455853156062688 ) ) ;
#38616=CARTESIAN_POINT ( 'NONE',  ( 1.363475323011903217, -276.5694342071035976, -206.1200871556967513 ) ) ;
#38617=CARTESIAN_POINT ( 'NONE',  ( 36.31276330658904072, -274.3841859489003241, -290.7476668553790091 ) ) ;
#38619=CARTESIAN_POINT ( 'NONE',  ( -107.9049296566723370, -290.0040694346157579, -251.0367197821137779 ) ) ;
#38621=CARTESIAN_POINT ( 'NONE',  ( -85.44268468821064744, -284.7553845316572279, -210.3643841496721905 ) ) ;
#38622=CARTESIAN_POINT ( 'NONE',  ( 32.02780294839854491, -279.4508296564083594, -244.4099689832119680 ) ) ;
#38623=CARTESIAN_POINT ( 'NONE',  ( 0.7201297632527839943, -279.1447965278727565, -207.3206021567679613 ) ) ;
#38624=CARTESIAN_POINT ( 'NONE',  ( -92.57354282915400745, -283.3336680961187994, -220.3779152993751040 ) ) ;
#38625=CARTESIAN_POINT ( 'NONE',  ( 32.81139473946547724, -289.8985705205326440, -297.0293547073904392 ) ) ;
#38626=CARTESIAN_POINT ( 'NONE',  ( -14.19814532920398698, -281.5640459856916209, -200.6546363802687836 ) ) ;
#38628=CARTESIAN_POINT ( 'NONE',  ( 1.666915929396587615, -280.9395187050885170, -335.8192594806904481 ) ) ;
#38629=CARTESIAN_POINT ( 'NONE',  ( -0.4212548499765729759, -296.5615698023182745, -335.6589921517457356 ) ) ;
#38630=CARTESIAN_POINT ( 'NONE',  ( -101.0294958830999121, -277.3447172651430037, -228.8191301985502548 ) ) ;
#38631=CARTESIAN_POINT ( 'NONE',  ( -106.3576983774112961, -278.8816436057744568, -294.6119849276227569 ) ) ;
#38632=CARTESIAN_POINT ( 'NONE',  ( -111.6783332568231515, -286.6994352809491602, -258.8774037793710363 ) ) ;
#38634=CARTESIAN_POINT ( 'NONE',  ( -44.78008781273001659, -293.8789889077572752, -195.1162027618132981 ) ) ;
#38635=CARTESIAN_POINT ( 'NONE',  ( 13.07378181987813370, -274.3481182185060447, -325.9588569955002981 ) ) ;
#38636=CARTESIAN_POINT ( 'NONE',  ( -70.57849786070354980, -288.6763976030566710, -339.6538109728577979 ) ) ;
#38637=CARTESIAN_POINT ( 'NONE',  ( 0.3348002583417372113, -290.9629698883056790, -206.9030867035255312 ) ) ;
#38639=CARTESIAN_POINT ( 'NONE',  ( -9.819120768379779207, -275.3698294393476544, -338.5198477838853819 ) ) ;
#38640=CARTESIAN_POINT ( 'NONE',  ( -109.1706596917610312, -294.4477471526549834, -289.1588678978764619 ) ) ;
#38641=CARTESIAN_POINT ( 'NONE',  ( -110.6128789897929323, -291.7844186261513073, -276.6889256733211937 ) ) ;
#38644=CARTESIAN_POINT ( 'NONE',  ( 24.26622432538682972, -291.4288702456225906, -225.3369977970235993 ) ) ;
#38645=CARTESIAN_POINT ( 'NONE',  ( 30.16500051966891860, -289.5507427126352695, -300.3088815223756001 ) ) ;
#38646=CARTESIAN_POINT ( 'NONE',  ( -70.22116375973402569, -287.7192440014742942, -338.8802677910119883 ) ) ;
#38647=CARTESIAN_POINT ( 'NONE',  ( -4.346509843980319587, -287.9211802676148864, -204.5835204515061037 ) ) ;
#38648=CARTESIAN_POINT ( 'NONE',  ( 22.88863428956209489, -288.9323752687214437, -311.9152228436436758 ) ) ;
#38649=CARTESIAN_POINT ( 'NONE',  ( -44.61130307516486937, -297.1234672522799656, -345.4171139492346470 ) ) ;
#38651=CARTESIAN_POINT ( 'NONE',  ( 37.12207665703658677, -288.9838700175615145, -288.3930817483354190 ) ) ;
#38652=CARTESIAN_POINT ( 'NONE',  ( -106.2726687366604637, -276.2277571832603940, -301.4374477890178241 ) ) ;
#38653=CARTESIAN_POINT ( 'NONE',  ( -113.2776127247878435, -278.7274505345936859, -282.9897152781234126 ) ) ;
#38654=CARTESIAN_POINT ( 'NONE',  ( -11.51245073006420583, -280.0461568319328762, -197.7889850670143517 ) ) ;
#38655=CARTESIAN_POINT ( 'NONE',  ( -80.70355945091367289, -299.4405467869611357, -209.6026127663645582 ) ) ;
#38656=CARTESIAN_POINT ( 'NONE',  ( -30.31933086257789611, -284.1406878904389828, -195.6384040962100244 ) ) ;
#38657=CARTESIAN_POINT ( 'NONE',  ( -110.3467704370464162, -272.3479781978851975, -270.3585183588572818 ) ) ;
#38658=CARTESIAN_POINT ( 'NONE',  ( -90.33908292914283322, -277.4323932189788025, -218.3061529871104369 ) ) ;
#38659=CARTESIAN_POINT ( 'NONE',  ( -44.26075426774872312, -281.1393677263657196, -345.0932572550127020 ) ) ;
#38661=CARTESIAN_POINT ( 'NONE',  ( 36.21208490114274525, -274.2893516052154723, -290.7210815904421679 ) ) ;
#38662=CARTESIAN_POINT ( 'NONE',  ( -107.3716679629555273, -298.3758536211280443, -247.2533725726121361 ) ) ;
#38663=CARTESIAN_POINT ( 'NONE',  ( 30.79618817293042454, -280.9280018609353533, -305.5565819910685263 ) ) ;
#38664=CARTESIAN_POINT ( 'NONE',  ( -65.67477836797526436, -298.6135027230203605, -202.8285693414526065 ) ) ;
#38665=CARTESIAN_POINT ( 'NONE',  ( -111.1120349551615476, -297.6116580182963389, -290.6400719286995127 ) ) ;
#38666=CARTESIAN_POINT ( 'NONE',  ( -76.57201217955358175, -273.1779267779495513, -208.7732124890071930 ) ) ;
#38667=CARTESIAN_POINT ( 'NONE',  ( 35.05375967640134149, -295.8047943575637078, -290.0033275576636242 ) ) ;
#38668=CARTESIAN_POINT ( 'NONE',  ( 7.542208665356192832, -286.8121861495543499, -207.7300053287800097 ) ) ;
#38669=CARTESIAN_POINT ( 'NONE',  ( -87.94853297784503354, -277.4307384113761827, -214.2517367298578108 ) ) ;
#38670=CARTESIAN_POINT ( 'NONE',  ( -87.38604648872859570, -289.5607974249431891, -328.9509221560660990 ) ) ;
#38671=CARTESIAN_POINT ( 'NONE',  ( -72.48226097449756367, -288.5882362391677134, -334.6149072242307057 ) ) ;
#38672=CARTESIAN_POINT ( 'NONE',  ( 16.08330946055215449, -290.8091783401737871, -217.6498664896715241 ) ) ;
#38674=CARTESIAN_POINT ( 'NONE',  ( -110.5532707284312579, -275.4615312476335589, -297.1751512281608143 ) ) ;
#38675=CARTESIAN_POINT ( 'NONE',  ( -8.199706663469738643, -288.1677005902176916, -337.4132053195290837 ) ) ;
#38677=CARTESIAN_POINT ( 'NONE',  ( -103.8426355183811864, -285.9946138933723319, -231.9089900136957567 ) ) ;
#38678=CARTESIAN_POINT ( 'NONE',  ( -7.271291010711933289, -291.4957559357231389, -199.7168827661001274 ) ) ;
#38679=CARTESIAN_POINT ( 'NONE',  ( 38.38554519050750002, -283.0044473123373336, -281.2552718805810059 ) ) ;
#38680=CARTESIAN_POINT ( 'NONE',  ( -95.92301247436604683, -283.7745094956986804, -313.9183200083140832 ) ) ;
#38681=CARTESIAN_POINT ( 'NONE',  ( -113.7747802549455542, -296.6687933634794945, -261.0345825958070236 ) ) ;
#38682=CARTESIAN_POINT ( 'NONE',  ( 24.19734696805935315, -276.3143142766277833, -230.1841449704854767 ) ) ;
#38683=CARTESIAN_POINT ( 'NONE',  ( 35.83380259722154193, -291.3821328833099074, -255.6236620708110081 ) ) ;
#38684=CARTESIAN_POINT ( 'NONE',  ( 23.38946471719789955, -273.7767295388932780, -229.1213853654839738 ) ) ;
#38687=CARTESIAN_POINT ( 'NONE',  ( -86.69887201954509237, -287.2802636248009662, -214.5680261316118447 ) ) ;
#38688=CARTESIAN_POINT ( 'NONE',  ( -74.44471193628359629, -296.6129916539582041, -337.5388327397262174 ) ) ;
#38689=CARTESIAN_POINT ( 'NONE',  ( -106.2670671519107373, -284.8780962609328640, -294.8672251754564968 ) ) ;
#38690=CARTESIAN_POINT ( 'NONE',  ( 37.94924438709335845, -274.7986959810210692, -285.3308837687211508 ) ) ;
#38691=CARTESIAN_POINT ( 'NONE',  ( -7.237762732274443778, -293.0881638256530550, -199.5861932270677528 ) ) ;
#38692=CARTESIAN_POINT ( 'NONE',  ( 23.72202852916559124, -285.0863190528654627, -225.5110731105860111 ) ) ;
#38693=CARTESIAN_POINT ( 'NONE',  ( 38.33724818304983017, -294.0625476862454661, -284.5192739322165494 ) ) ;
#38694=CARTESIAN_POINT ( 'NONE',  ( -106.0510309508754290, -290.5562900909282575, -295.0818652329948009 ) ) ;
#38697=CARTESIAN_POINT ( 'NONE',  ( -47.07807668347071939, -155.4490103796987626, -361.3962506754892843 ) ) ;
#38698=CARTESIAN_POINT ( 'NONE',  ( -111.5403815227015087, -285.8467827904743785, -288.2282632799791600 ) ) ;
#38699=CARTESIAN_POINT ( 'NONE',  ( -2.602324593224659921, -271.9809262143061233, -198.2974183793908196 ) ) ;
#38700=VERTEX_POINT ( 'NONE', #34482 ) ;
#38701=CARTESIAN_POINT ( 'NONE',  ( -97.79501939187794335, -282.8966276932354162, -311.9179422820130867 ) ) ;
#38702=CARTESIAN_POINT ( 'NONE',  ( -114.0584231396461945, -278.1317557054591134, -277.3249408792123063 ) ) ;
#38703=CARTESIAN_POINT ( 'NONE',  ( 17.17859992772618583, -284.2728057876785215, -321.6956901318080781 ) ) ;
#38704=CARTESIAN_POINT ( 'NONE',  ( -45.94015373935981472, -156.1293870317898893, -363.6621071055034804 ) ) ;
#38705=CARTESIAN_POINT ( 'NONE',  ( -50.01380106442190510, -281.7853987947431733, -345.7672475420787919 ) ) ;
#38706=CARTESIAN_POINT ( 'NONE',  ( 36.75393891632501209, -285.6888538904835286, -279.3989870114871223 ) ) ;
#38707=CARTESIAN_POINT ( 'NONE',  ( -85.04911771501511453, -275.2620658605604831, -211.5027474227059372 ) ) ;
#38708=CARTESIAN_POINT ( 'NONE',  ( -70.95353362183402623, -296.0005070196287988, -335.2460091929279997 ) ) ;
#38709=CARTESIAN_POINT ( 'NONE',  ( -37.53454268933070637, -290.7345485004443617, -196.8556903180865163 ) ) ;
#38710=CARTESIAN_POINT ( 'NONE',  ( -103.3283961143731489, -279.7202660643321224, -230.7725192632215681 ) ) ;
#38711=CARTESIAN_POINT ( 'NONE',  ( -8.738677133535908581, -276.6671966870574693, -337.5376493299509093 ) ) ;
#38712=CARTESIAN_POINT ( 'NONE',  ( 38.82888932785649416, -274.5900494434139318, -279.7238603916275679 ) ) ;
#38714=CARTESIAN_POINT ( 'NONE',  ( 35.97090622290477313, -273.7558361698543195, -286.2401664282711522 ) ) ;
#38715=CARTESIAN_POINT ( 'NONE',  ( 31.70542278211600262, -295.4014500383208315, -303.2122022881757744 ) ) ;
#38719=CARTESIAN_POINT ( 'NONE',  ( -78.53903684522647666, -284.7011510993472712, -330.9994352447401411 ) ) ;
#38720=CARTESIAN_POINT ( 'NONE',  ( -38.69176861510950971, -284.8290019289717065, -346.3357935782334494 ) ) ;
#38721=CARTESIAN_POINT ( 'NONE',  ( -19.78335102989808902, -285.6325094345863818, -199.3991771637086003 ) ) ;
#38722=CARTESIAN_POINT ( 'NONE',  ( 29.87460138361937823, -274.3582520091341621, -300.8309263861464160 ) ) ;
#38723=CARTESIAN_POINT ( 'NONE',  ( 35.70506315066613467, -283.5851191530240953, -283.6625824098250632 ) ) ;
#38724=CARTESIAN_POINT ( 'NONE',  ( -24.22503359630115582, -275.3616467007357755, -342.9296799161996319 ) ) ;
#38725=CARTESIAN_POINT ( 'NONE',  ( -13.67264448623344641, -277.8173867107839214, -339.7974934417040913 ) ) ;
#38726=CARTESIAN_POINT ( 'NONE',  ( 121.3395553409046528, -299.5541904835127980, -198.8526868767648352 ) ) ;
#38728=CARTESIAN_POINT ( 'NONE',  ( -11.57315864699415542, -281.1820874616586252, -197.9164376734674704 ) ) ;
#38729=CARTESIAN_POINT ( 'NONE',  ( -39.59174666557483846, -280.5169852378463133, -193.4425240798844072 ) ) ;
#38733=CARTESIAN_POINT ( 'NONE',  ( 35.49703938673690828, -289.1447596469518544, -249.3226175423496898 ) ) ;
#38734=CARTESIAN_POINT ( 'NONE',  ( -84.17036566300784273, -296.5863989790245228, -214.0839696217804828 ) ) ;
#38736=CARTESIAN_POINT ( 'NONE',  ( -97.37877477793637127, -290.5452482676105888, -222.3104941083730637 ) ) ;
#38737=CARTESIAN_POINT ( 'NONE',  ( 36.37445050113649359, -286.0052496041078598, -268.3123165637961733 ) ) ;
#38738=CARTESIAN_POINT ( 'NONE',  ( -39.99741367048822127, -287.6607675278536931, -343.9523932668482757 ) ) ;
#38739=CARTESIAN_POINT ( 'NONE',  ( -95.90260588986973289, -289.4205672298264744, -225.0997179538059640 ) ) ;
#38740=CARTESIAN_POINT ( 'NONE',  ( -87.97948325793061031, -286.5295761286000698, -217.2297202608392865 ) ) ;
#38741=CARTESIAN_POINT ( 'NONE',  ( -89.94493109208984549, -275.7943569993038864, -323.8932079826837480 ) ) ;
#38742=CARTESIAN_POINT ( 'NONE',  ( 23.49111873604502776, -286.5695375880597453, -316.2502078246037627 ) ) ;
#38743=CARTESIAN_POINT ( 'NONE',  ( 32.00032400169781255, -289.1778863366087080, -241.6478666014458270 ) ) ;
#38744=CARTESIAN_POINT ( 'NONE',  ( -6.404888942851536093, -286.6465964779599744, -338.8661699398362543 ) ) ;
#38746=CARTESIAN_POINT ( 'NONE',  ( 34.71911799381504693, -282.6661037326872474, -283.4946402849566311 ) ) ;
#38747=CARTESIAN_POINT ( 'NONE',  ( -109.7684818101180610, -292.2942188605396723, -290.4705616292967534 ) ) ;
#38750=CARTESIAN_POINT ( 'NONE',  ( -54.29627683302920360, -299.7561801430052810, -196.7278610676924302 ) ) ;
#38751=CARTESIAN_POINT ( 'NONE',  ( 5.024963202835075471, -279.8386635464007099, -210.7149314764068890 ) ) ;
#38752=CARTESIAN_POINT ( 'NONE',  ( 35.88783707607991147, -279.7599993690577094, -286.5609801482431180 ) ) ;
#38753=CARTESIAN_POINT ( 'NONE',  ( 24.74974782781754001, -293.3516067526378492, -315.6470700573532895 ) ) ;
#38754=CARTESIAN_POINT ( 'NONE',  ( -44.62801135734449787, -296.3584260429999517, -196.8707527219877704 ) ) ;
#38755=CARTESIAN_POINT ( 'NONE',  ( -8.196989202679366926, -274.7473528729238978, -338.8723705916961535 ) ) ;
#38756=CARTESIAN_POINT ( 'NONE',  ( -58.53454759373760652, -296.6471662342117952, -340.7323244043890895 ) ) ;
#38758=CARTESIAN_POINT ( 'NONE',  ( -71.12582338760221035, -272.1896853246867636, -201.8247093305806743 ) ) ;
#38759=CARTESIAN_POINT ( 'NONE',  ( -112.3852040423190175, -294.9443124747785419, -258.3437437178201890 ) ) ;
#38760=CARTESIAN_POINT ( 'NONE',  ( 11.30684363273117299, -294.1669617081450951, -215.0781558697165963 ) ) ;
#38762=CARTESIAN_POINT ( 'NONE',  ( -7.213068811878641462, -293.2606274030360964, -203.6912799562599616 ) ) ;
#38764=CARTESIAN_POINT ( 'NONE',  ( -95.02781199097549347, -281.9050084632482367, -318.8653086749613408 ) ) ;
#38765=CARTESIAN_POINT ( 'NONE',  ( -20.84817480361739683, -294.8346421280153322, -341.5255537009674072 ) ) ;
#38766=CARTESIAN_POINT ( 'NONE',  ( -18.91839532270654090, -282.8214490829483339, -345.1795817661326851 ) ) ;
#38767=CARTESIAN_POINT ( 'NONE',  ( 12.03239917661917069, -282.6526394970497904, -213.1639807011012238 ) ) ;
#38768=CARTESIAN_POINT ( 'NONE',  ( -36.56138241309975001, -285.7284152807337136, -193.3731814531014379 ) ) ;
#38769=CARTESIAN_POINT ( 'NONE',  ( -104.0321345044617658, -289.0031135123950889, -236.2992576045764679 ) ) ;
#38770=CARTESIAN_POINT ( 'NONE',  ( 30.45221852812324315, -280.4876221868914286, -305.3852859837128904 ) ) ;
#38771=CARTESIAN_POINT ( 'NONE',  ( 9.356661063313353566, -285.3946019829459146, -213.6116110365334748 ) ) ;
#38772=CARTESIAN_POINT ( 'NONE',  ( -15.05526900853502070, -287.6905604449424914, -343.7978897630304118 ) ) ;
#38774=CARTESIAN_POINT ( 'NONE',  ( -82.83714306084179668, -297.2859992475754325, -328.5348221971021871 ) ) ;
#38775=CARTESIAN_POINT ( 'NONE',  ( -82.18570005214883167, -279.0760004505090137, -332.2288960437002174 ) ) ;
#38776=CARTESIAN_POINT ( 'NONE',  ( -11.64237395522665963, -292.7393832104152693, -341.2539716593892649 ) ) ;
#38777=CARTESIAN_POINT ( 'NONE',  ( -43.74871671564858389, -279.6358140187750223, -197.5713504666764209 ) ) ;
#38778=CARTESIAN_POINT ( 'NONE',  ( 33.32355502936599123, -293.3290886519993137, -239.7764532301270890 ) ) ;
#38779=CARTESIAN_POINT ( 'NONE',  ( -110.9512616473154907, -282.8493949467728044, -253.3039594950243725 ) ) ;
#38780=CARTESIAN_POINT ( 'NONE',  ( -41.25396738523028262, -279.1015408230006187, -345.2718797789061682 ) ) ;
#38781=CARTESIAN_POINT ( 'NONE',  ( -18.17041146242248928, -293.8576538703090932, -341.0425875367765798 ) ) ;
#38782=CARTESIAN_POINT ( 'NONE',  ( -69.83879782982727136, -295.6240379137856280, -202.7671885601548638 ) ) ;
#38785=CARTESIAN_POINT ( 'NONE',  ( 36.33091610447689135, -283.6869611531528790, -282.3691328587689213 ) ) ;
#38786=CARTESIAN_POINT ( 'NONE',  ( -109.4246530689027566, -295.9027183941707335, -282.2790178427223964 ) ) ;
#38788=CARTESIAN_POINT ( 'NONE',  ( -95.95921662488163406, -270.6952119285918457, -223.5744983911110353 ) ) ;
#38789=CARTESIAN_POINT ( 'NONE',  ( 98.67988849359637982, -298.7747639397677517, -193.6174340023339369 ) ) ;
#38790=CARTESIAN_POINT ( 'NONE',  ( 36.21242324690683034, -288.5996057745439884, -249.1234694261997049 ) ) ;
#38791=CARTESIAN_POINT ( 'NONE',  ( -72.36072668084190695, -289.3626830585199627, -334.4131888609855991 ) ) ;
#38792=CARTESIAN_POINT ( 'NONE',  ( -105.0869751600894659, -280.4582392001921107, -241.3561966493277282 ) ) ;
#38793=CARTESIAN_POINT ( 'NONE',  ( -47.43278820255034844, -299.6824456453469452, -196.9870020056213207 ) ) ;
#38794=CARTESIAN_POINT ( 'NONE',  ( -51.89114037787017963, -278.6568620729844952, -198.3685471001835765 ) ) ;
#38796=CARTESIAN_POINT ( 'NONE',  ( -14.81354312561614783, -297.9937060428184168, -193.3834923250184090 ) ) ;
#38797=CARTESIAN_POINT ( 'NONE',  ( -47.20907965767397485, -293.8459718442173312, -196.5779964881937190 ) ) ;
#38800=CARTESIAN_POINT ( 'NONE',  ( -75.91549562676297569, -290.2336861823890786, -332.4574541783235304 ) ) ;
#38802=CARTESIAN_POINT ( 'NONE',  ( 23.83137965190389096, -291.0886312732263264, -225.6603373111316273 ) ) ;
#38803=CARTESIAN_POINT ( 'NONE',  ( -98.46294381318374178, -296.7735133423636853, -230.3161378687463809 ) ) ;
#38805=CARTESIAN_POINT ( 'NONE',  ( -111.5835760717182694, -291.8490584600560283, -288.0479520807988365 ) ) ;
#38806=CARTESIAN_POINT ( 'NONE',  ( -99.90806341382572953, -287.6948066931273047, -220.5068182859052968 ) ) ;
#38807=CARTESIAN_POINT ( 'NONE',  ( 36.94720901235586297, -289.6682648504477129, -279.3714678376840084 ) ) ;
#38808=CARTESIAN_POINT ( 'NONE',  ( 32.97593397404876470, -273.8865216925588584, -296.1134837117195957 ) ) ;
#38809=CARTESIAN_POINT ( 'NONE',  ( 36.81036916302631568, -277.3804418757688381, -263.2595170955654567 ) ) ;
#38810=CARTESIAN_POINT ( 'NONE',  ( -4.169845387424268246, -290.5727406007346190, -203.7065217159041310 ) ) ;
#38811=CARTESIAN_POINT ( 'NONE',  ( -94.05320953328877920, -281.1042910461220572, -220.1205946689422603 ) ) ;
#38813=CARTESIAN_POINT ( 'NONE',  ( -56.35339028472269263, -282.6522753933383001, -340.9475777694492535 ) ) ;
#38814=CARTESIAN_POINT ( 'NONE',  ( -84.66479131761597898, -278.7662605811159438, -330.7777176819421356 ) ) ;
#38815=CARTESIAN_POINT ( 'NONE',  ( 13.40619459087050203, -281.1557541020961253, -327.8134145612160637 ) ) ;
#38816=CARTESIAN_POINT ( 'NONE',  ( 31.03526160566912040, -276.0426467268437705, -235.4696961664207322 ) ) ;
#38818=CARTESIAN_POINT ( 'NONE',  ( -38.36768189626314296, -275.5596251077748775, -194.0613465760981740 ) ) ;
#38819=CARTESIAN_POINT ( 'NONE',  ( -67.68488546085839630, -279.9805209788415823, -333.4427485647536855 ) ) ;
#38821=CARTESIAN_POINT ( 'NONE',  ( -106.8049319824969956, -298.1835524501046280, -298.6429154254506102 ) ) ;
#38822=CARTESIAN_POINT ( 'NONE',  ( -108.0201540150592905, -291.3735363975515611, -290.0103841145019601 ) ) ;
#38823=CARTESIAN_POINT ( 'NONE',  ( -57.00675063579810598, -291.0624103628849753, -343.8134480378828357 ) ) ;
#38824=CARTESIAN_POINT ( 'NONE',  ( -55.02900067885569513, -291.1672101448540388, -199.4312084446210633 ) ) ;
#38825=CARTESIAN_POINT ( 'NONE',  ( -91.85496449419646581, -284.8071997122972903, -216.0671872784213576 ) ) ;
#38827=CARTESIAN_POINT ( 'NONE',  ( 8.272607584459853669, -280.8163346047826963, -328.4416725878276679 ) ) ;
#38828=CARTESIAN_POINT ( 'NONE',  ( 1.985699335745167327, -290.3800937224756922, -333.3231790262706227 ) ) ;
#38829=CARTESIAN_POINT ( 'NONE',  ( -64.32711367824913395, -281.8907011518411423, -338.9358597490014517 ) ) ;
#38830=CARTESIAN_POINT ( 'NONE',  ( 35.84177963000056621, -282.7720054275216626, -263.0859850048537396 ) ) ;
#38831=CARTESIAN_POINT ( 'NONE',  ( 33.82870509269117321, -288.8613445592978906, -299.2706865993270071 ) ) ;
#38832=CARTESIAN_POINT ( 'NONE',  ( -76.86041000289702652, -279.9999044749450832, -208.8495236173278329 ) ) ;
#38833=CARTESIAN_POINT ( 'NONE',  ( 21.91192499489778100, -291.6917885894774258, -221.8120023364671169 ) ) ;
#38834=CARTESIAN_POINT ( 'NONE',  ( 29.98513318908628023, -287.8731388192978784, -233.2202653767533320 ) ) ;
#38835=CARTESIAN_POINT ( 'NONE',  ( -49.34132053080093527, -286.3955993419867241, -194.3104772342489355 ) ) ;
#38836=CARTESIAN_POINT ( 'NONE',  ( -95.11513802396738981, -284.0903345210262501, -315.0047211613770628 ) ) ;
#38839=CARTESIAN_POINT ( 'NONE',  ( 20.35418469003431952, -294.7394456007099848, -221.2343779958318351 ) ) ;
#38840=CARTESIAN_POINT ( 'NONE',  ( 37.58239763731098293, -292.0413089025782938, -254.8153091839437252 ) ) ;
#38841=CARTESIAN_POINT ( 'NONE',  ( -56.67378824133316328, -276.3661706069784714, -341.0514464796813172 ) ) ;
#38842=CARTESIAN_POINT ( 'NONE',  ( -23.37448629464264016, -297.5713107977072696, -193.4645463883891523 ) ) ;
#38843=CARTESIAN_POINT ( 'NONE',  ( 21.55952134324993708, -291.4160008093153920, -226.0739430527690104 ) ) ;
#38844=CARTESIAN_POINT ( 'NONE',  ( -99.28351402288689087, -295.3468833874654820, -229.7568633292858635 ) ) ;
#38845=CARTESIAN_POINT ( 'NONE',  ( -12.13819365048166432, -293.5924916550139869, -201.3728256543343775 ) ) ;
#38846=CARTESIAN_POINT ( 'NONE',  ( 6.851689802359501869, -293.7495103260690712, -211.8703464102424618 ) ) ;
#38847=CARTESIAN_POINT ( 'NONE',  ( -6.572041688988396579, -292.6488985891979837, -338.9414107010813382 ) ) ;
#38849=CARTESIAN_POINT ( 'NONE',  ( 1.446330167486975293, -289.4610779507010534, -332.4811401472002785 ) ) ;
#38850=CARTESIAN_POINT ( 'NONE',  ( -68.31574903800111542, -279.4368442109777675, -339.0703002293935810 ) ) ;
#38851=CARTESIAN_POINT ( 'NONE',  ( -35.73530157983303468, -275.8273832322307157, -346.9602576719697140 ) ) ;
#38853=CARTESIAN_POINT ( 'NONE',  ( -90.08690079926110172, -272.6789446726293704, -214.3307775404495032 ) ) ;
#38854=CARTESIAN_POINT ( 'NONE',  ( 35.34123567665463383, -279.8399928478545462, -286.4392100515612469 ) ) ;
#38855=CARTESIAN_POINT ( 'NONE',  ( -64.82574785959964458, -275.8049203512368308, -341.4876891502080412 ) ) ;
#38857=CARTESIAN_POINT ( 'NONE',  ( -88.85940884276104157, -294.4788143193874816, -322.8460981224324087 ) ) ;
#38859=CARTESIAN_POINT ( 'NONE',  ( -105.5143021396919352, -273.5573520494992295, -243.8322591845377758 ) ) ;
#38861=CARTESIAN_POINT ( 'NONE',  ( -105.0470168024887982, -288.1368325642215495, -303.5614767484809704 ) ) ;
#38862=CARTESIAN_POINT ( 'NONE',  ( -4.102791441679141116, -274.3364638657860155, -205.3534317641578753 ) ) ;
#38863=CARTESIAN_POINT ( 'NONE',  ( -8.233132333283057491, -288.6813746547723554, -341.6613665754782687 ) ) ;
#38864=CARTESIAN_POINT ( 'NONE',  ( -111.2699889068196057, -274.7299603236163534, -256.4946206855208857 ) ) ;
#38865=CARTESIAN_POINT ( 'NONE',  ( -98.36330645575226583, -295.1420787051656589, -227.0437774687291324 ) ) ;
#38866=CARTESIAN_POINT ( 'NONE',  ( -37.32457320118455613, -282.2490785764852603, -347.2126780741660923 ) ) ;
#38867=DIRECTION ( 'NONE',  ( 0.000000000000000000, 0.000000000000000000, -1.000000000000000000 ) ) ;
#38868=CARTESIAN_POINT ( 'NONE',  ( -78.41963187038422234, -281.6043709599552471, -333.1727363578929157 ) ) ;
#38870=CARTESIAN_POINT ( 'NONE',  ( -91.95842277358480032, -290.0452186496872287, -221.3102519504354575 ) ) ;
#38871=CARTESIAN_POINT ( 'NONE',  ( -34.82805275105177145, -281.1598582553121446, -344.5664000865866115 ) ) ;
#38873=CARTESIAN_POINT ( 'NONE',  ( -101.4071529614679150, -289.0747590817246078, -231.3660105916091254 ) ) ;
#38874=CARTESIAN_POINT ( 'NONE',  ( -83.64107105132380582, -274.9235214554420850, -213.0280908289012416 ) ) ;
#38875=CARTESIAN_POINT ( 'NONE',  ( -34.47836883863266166, -284.2219802332732002, -346.9105141488691402 ) ) ;
#38876=CARTESIAN_POINT ( 'NONE',  ( -70.74381144164148338, -271.6948836715877746, -202.5849189003282333 ) ) ;
#38877=CARTESIAN_POINT ( 'NONE',  ( -71.40888074852966838, -283.5153415121228022, -334.9244760471290761 ) ) ;
#38878=CARTESIAN_POINT ( 'NONE',  ( 34.94896151333151835, -276.7973176353905274, -256.5975734602923808 ) ) ;
#38879=CARTESIAN_POINT ( 'NONE',  ( -4.985487101250802411, -277.4177748106638433, -335.9926991493922515 ) ) ;
#38880=CARTESIAN_POINT ( 'NONE',  ( -69.58654837798279402, -285.4766549964556361, -338.0898269894869941 ) ) ;
#38882=CARTESIAN_POINT ( 'NONE',  ( -111.5368827832384255, -270.7108482962777316, -270.3376737736280120 ) ) ;
#38883=CARTESIAN_POINT ( 'NONE',  ( 11.19666648565100786, -294.2346486981763860, -330.2046296897908633 ) ) ;
#38884=CARTESIAN_POINT ( 'NONE',  ( -8.889260789513871330, -288.4060450473700143, -201.3378485982815675 ) ) ;
#38886=CARTESIAN_POINT ( 'NONE',  ( -99.90806341382575795, -287.4094976428775112, -320.2154176792147382 ) ) ;
#38887=CARTESIAN_POINT ( 'NONE',  ( -48.06191697002892482, -278.8392922549081732, -194.3695591657247803 ) ) ;
#38888=CARTESIAN_POINT ( 'NONE',  ( -96.82614518502526835, -289.5966867193443477, -222.7371616665716374 ) ) ;
#38889=CARTESIAN_POINT ( 'NONE',  ( -49.55532178199268856, -287.4138687008414195, -197.6349567661305002 ) ) ;
#38890=CARTESIAN_POINT ( 'NONE',  ( -4.597880586798756219, -278.3749284970634790, -336.7515262305816464 ) ) ;
#38891=CARTESIAN_POINT ( 'NONE',  ( -98.88057810649675616, -286.5847806301068204, -224.9797424687994862 ) ) ;
#38892=CARTESIAN_POINT ( 'NONE',  ( 37.42496333949119247, -283.6362855124600628, -276.9008602133670820 ) ) ;
#38893=CARTESIAN_POINT ( 'NONE',  ( 39.13784383678476075, -275.8361999596876331, -279.7457900415583936 ) ) ;
#38894=CARTESIAN_POINT ( 'NONE',  ( -112.1750334612222417, -270.5523135732584024, -270.3357091355649118 ) ) ;
#38895=CARTESIAN_POINT ( 'NONE',  ( -114.2321197488982563, -278.3341150095947114, -274.4676219728029309 ) ) ;
#38896=CARTESIAN_POINT ( 'NONE',  ( -69.90918191436207962, -299.5399602978421285, -203.4232861379292672 ) ) ;
#38899=CARTESIAN_POINT ( 'NONE',  ( -96.36887887570836142, -295.3387268779783881, -222.8627216518738123 ) ) ;
#38900=FACE_OUTER_BOUND ( 'NONE', #19360, .T. ) ;
#38901=CARTESIAN_POINT ( 'NONE',  ( -109.9659129573688716, -277.9486957903625353, -278.7906956079009433 ) ) ;
#38902=CARTESIAN_POINT ( 'NONE',  ( 26.59067294840640017, -276.1994243524819694, -228.1632461027326428 ) ) ;
#38903=CARTESIAN_POINT ( 'NONE',  ( -0.4989284012178738514, -281.6335584687190021, -337.7216144051529341 ) ) ;
#38904=CARTESIAN_POINT ( 'NONE',  ( 10.79103590186578288, -290.1364750279996088, -326.6535731360902446 ) ) ;
#38905=CARTESIAN_POINT ( 'NONE',  ( -101.0387348915883479, -297.5136553189619804, -312.4732526350452986 ) ) ;
#38906=CARTESIAN_POINT ( 'NONE',  ( -74.40074275643280544, -296.7383757356394653, -337.4625644740273742 ) ) ;
#38907=CARTESIAN_POINT ( 'NONE',  ( 29.10296112272665425, -295.0955987878288056, -235.9353222072598726 ) ) ;
#38908=CARTESIAN_POINT ( 'NONE',  ( 25.22910672298099044, -278.9957808248648803, -229.2198148158289541 ) ) ;
#38909=CARTESIAN_POINT ( 'NONE',  ( 34.84613560998990067, -283.2365130819293313, -252.1371520393899175 ) ) ;
#38910=CARTESIAN_POINT ( 'NONE',  ( -98.04308173675568128, -295.2220722057135731, -227.2721812352086772 ) ) ;
#38911=CARTESIAN_POINT ( 'NONE',  ( -107.2009437233996891, -286.5458036563655924, -239.7967779330370774 ) ) ;
#38912=CARTESIAN_POINT ( 'NONE',  ( 32.60441912591705460, -286.7641590877215663, -292.4791470319245832 ) ) ;
#38913=CARTESIAN_POINT ( 'NONE',  ( 27.76947042884798122, -280.3632157620247085, -229.3486196732935127 ) ) ;
#38914=CARTESIAN_POINT ( 'NONE',  ( -46.31138446648969165, -155.9421665903751659, -364.5751334320801789 ) ) ;
#38916=CARTESIAN_POINT ( 'NONE',  ( 20.11773611681064011, -286.8138030240005492, -320.7496581208525299 ) ) ;
#38917=CARTESIAN_POINT ( 'NONE',  ( -41.31983851173026778, -285.6674403338118395, -197.4359154329331716 ) ) ;
#38919=CARTESIAN_POINT ( 'NONE',  ( -47.20294258024109979, -284.2543210959161684, -346.4153644551080902 ) ) ;
#38920=CARTESIAN_POINT ( 'NONE',  ( 33.60808501386378566, -276.1138442194991285, -287.6827196816861374 ) ) ;
#38921=CARTESIAN_POINT ( 'NONE',  ( -79.41330786547507614, -290.4190967844235729, -206.1768812656930834 ) ) ;
#38922=CARTESIAN_POINT ( 'NONE',  ( 34.22650671086350371, -281.8448330589279180, -242.0856870232992151 ) ) ;
#38924=CARTESIAN_POINT ( 'NONE',  ( -98.03675291034157624, -280.6945823384134542, -224.0924663166605910 ) ) ;
#38925=CARTESIAN_POINT ( 'NONE',  ( 31.06029978177634732, -282.3407270155029778, -305.6727407117599569 ) ) ;
#38926=CARTESIAN_POINT ( 'NONE',  ( -53.35057174420112602, -286.7666405000204577, -340.3538533559490702 ) ) ;
#38927=CARTESIAN_POINT ( 'NONE',  ( 154.5379790899321222, 206.7802150222307205, -217.4094443645867614 ) ) ;
#38929=CARTESIAN_POINT ( 'NONE',  ( 26.83531001496087143, -277.0346737873732650, -231.7726260706255630 ) ) ;
#38930=CARTESIAN_POINT ( 'NONE',  ( -110.6672959571649102, -266.1490546199543701, -306.8034369765820202 ) ) ;
#38931=CARTESIAN_POINT ( 'NONE',  ( 36.19165312914957155, -279.4066972170023178, -257.5278501546050052 ) ) ;
#38932=CARTESIAN_POINT ( 'NONE',  ( -103.8078168060792308, -296.3120501644810361, -239.8066296507456912 ) ) ;
#38933=CARTESIAN_POINT ( 'NONE',  ( 22.23499882974141073, -293.7140350553862049, -319.0659211555440606 ) ) ;
#38934=CARTESIAN_POINT ( 'NONE',  ( -101.6167628974845485, -254.6067659492810549, -324.2419241925626920 ) ) ;
#38935=CARTESIAN_POINT ( 'NONE',  ( 97.90671567993493341, -298.2887776826660797, -193.9822965058080513 ) ) ;
#38936=CARTESIAN_POINT ( 'NONE',  ( -80.89588987942693166, -288.0539845580580618, -330.0021757292981874 ) ) ;
#38937=CARTESIAN_POINT ( 'NONE',  ( -39.70502066771997107, -296.9425305464727671, -344.5713344866962871 ) ) ;
#38938=CARTESIAN_POINT ( 'NONE',  ( 20.72002864524939980, -288.2369376787176520, -225.3047185328026103 ) ) ;
#38940=CARTESIAN_POINT ( 'NONE',  ( 6.352435600664771975, -293.5711424186819158, -207.2450129433816812 ) ) ;
#38941=CARTESIAN_POINT ( 'NONE',  ( -95.81896027629571222, -285.6587821465279262, -226.5615918734511069 ) ) ;
#38942=CARTESIAN_POINT ( 'NONE',  ( -113.8715407284473997, -271.5443771474579648, -264.6355703682659168 ) ) ;
#38943=CARTESIAN_POINT ( 'NONE',  ( -70.83657853913591396, -292.4242929471875527, -201.2072898770309450 ) ) ;
#38944=CARTESIAN_POINT ( 'NONE',  ( -40.63606544407501531, -292.5041375600537776, -193.4800462869531543 ) ) ;
#38945=CARTESIAN_POINT ( 'NONE',  ( -102.8444971011521716, -290.2821861333493985, -302.5850779066218479 ) ) ;
#38948=CARTESIAN_POINT ( 'NONE',  ( -15.28277488989663091, -300.1859184509785905, -194.5894067391707836 ) ) ;
#38949=CARTESIAN_POINT ( 'NONE',  ( -99.23710006424150265, -271.9502294218637530, -225.1403997163347697 ) ) ;
#38950=CARTESIAN_POINT ( 'NONE',  ( -8.412290636039669423, -281.7226062797830082, -337.6403697251629410 ) ) ;
#38952=CARTESIAN_POINT ( 'NONE',  ( 10.48289776478432067, -275.9198106377223780, -330.6979981948464342 ) ) ;
#38953=CARTESIAN_POINT ( 'NONE',  ( -57.05592824709768252, -272.1935891791212043, -199.1896894604461465 ) ) ;
#38954=CARTESIAN_POINT ( 'NONE',  ( -96.61202424024402546, -281.0301961139024343, -225.6422002244793532 ) ) ;
#38955=CARTESIAN_POINT ( 'NONE',  ( 16.47733404406061908, -274.4165876544465164, -321.4920972521829299 ) ) ;
#38956=CARTESIAN_POINT ( 'NONE',  ( -93.92948339625232279, -298.4164489833885909, -223.5980776592406869 ) ) ;
#38957=CARTESIAN_POINT ( 'NONE',  ( 52.12983541473749227, -300.2777557423787016, -197.0351508630318449 ) ) ;
#38958=CARTESIAN_POINT ( 'NONE',  ( -111.5005418464798623, -298.3736825558245869, -252.8423676410268115 ) ) ;
#38959=CARTESIAN_POINT ( 'NONE',  ( -38.31042497412869352, -272.0601773622864243, -195.0121406894418215 ) ) ;
#38960=CARTESIAN_POINT ( 'NONE',  ( 33.40476224272852335, -293.9608878124998910, -251.9537626458941304 ) ) ;
#38961=CARTESIAN_POINT ( 'NONE',  ( 9.235706666057446057, -291.2808837788294340, -213.3220331965499952 ) ) ;
#38963=CARTESIAN_POINT ( 'NONE',  ( -42.79554508842491600, -277.6115874670767312, -347.1060362404298303 ) ) ;
#38964=CARTESIAN_POINT ( 'NONE',  ( -40.52313901784983585, -298.3443636269313970, -197.3967600650562133 ) ) ;
#38965=CARTESIAN_POINT ( 'NONE',  ( -47.20945034132956408, -281.8598615415051540, -346.2289357820915825 ) ) ;
#38966=CARTESIAN_POINT ( 'NONE',  ( 29.28925649795061048, -296.0120784328213404, -305.1511171591659490 ) ) ;
#38968=CARTESIAN_POINT ( 'NONE',  ( -48.36307516380174576, -282.3931924909401232, -342.6876761677719401 ) ) ;
#38969=CARTESIAN_POINT ( 'NONE',  ( -112.4925948611060278, -282.5929181930020491, -267.1663043245724793 ) ) ;
#38971=CARTESIAN_POINT ( 'NONE',  ( -1.196520178436188742, -275.1376827105027019, -334.5194833867844295 ) ) ;
#38972=CARTESIAN_POINT ( 'NONE',  ( 16.94890696751424741, -282.8253361369538652, -218.5421941955870011 ) ) ;
#38975=CARTESIAN_POINT ( 'NONE',  ( -95.40473791851191265, -271.6244640803246853, -220.9940584642222348 ) ) ;
#38976=CARTESIAN_POINT ( 'NONE',  ( -109.5825018052297963, -280.8190351038822996, -249.5934748548683331 ) ) ;
#38978=CARTESIAN_POINT ( 'NONE',  ( -5.405234742231955103, -288.3891990309886069, -201.8820965183122382 ) ) ;
#38979=CARTESIAN_POINT ( 'NONE',  ( -105.9330854110499445, -288.1531488174302353, -300.8227834273016015 ) ) ;
#38980=DIRECTION ( 'NONE',  ( -1.000000000000000000, -0.000000000000000000, -0.000000000000000000 ) ) ;
#38981=CARTESIAN_POINT ( 'NONE',  ( -73.51137206751494091, -294.3385038110995424, -334.2272697142782363 ) ) ;
#38982=CARTESIAN_POINT ( 'NONE',  ( -42.77762028594852950, -287.2609067412499257, -344.4484903202602482 ) ) ;
#38983=CARTESIAN_POINT ( 'NONE',  ( -96.00709874043252512, -235.9016261432062720, -336.2420922186948928 ) ) ;
#38984=CARTESIAN_POINT ( 'NONE',  ( -109.7603545548370931, -294.8033588189083503, -250.8042810271120402 ) ) ;
#38985=CARTESIAN_POINT ( 'NONE',  ( 38.94730303222441847, -286.0113107290040375, -268.7192447469402623 ) ) ;
#38986=CARTESIAN_POINT ( 'NONE',  ( 5.369751610799484709, -282.2412376619672045, -210.1766324091266824 ) ) ;
#38987=CARTESIAN_POINT ( 'NONE',  ( -35.94065552927719409, -281.2747063901879301, -346.3478152406299841 ) ) ;
#38988=CARTESIAN_POINT ( 'NONE',  ( -5.792432161130517621, -288.6253538558429454, -336.1915341345905972 ) ) ;
#38989=CARTESIAN_POINT ( 'NONE',  ( 15.67135945481114234, -282.2456455428496156, -219.2492358807538153 ) ) ;
#38990=CARTESIAN_POINT ( 'NONE',  ( -5.954411318788324969, -283.4315928472718156, -336.4615079754016733 ) ) ;
#38991=CARTESIAN_POINT ( 'NONE',  ( 37.46108697011733568, -289.6538132388272970, -279.8896436220896931 ) ) ;
#38992=CARTESIAN_POINT ( 'NONE',  ( -14.81224999962049438, -298.4936074059563680, -193.3604978767456544 ) ) ;
#38994=CARTESIAN_POINT ( 'NONE',  ( -36.93973224474150641, -274.0570866927869815, -193.3491151106246946 ) ) ;
#38995=CARTESIAN_POINT ( 'NONE',  ( -36.20583416707631130, -294.0463177621254545, -195.7121984873012366 ) ) ;
#38997=CARTESIAN_POINT ( 'NONE',  ( -69.85430415644619018, -285.9805209788416391, -337.9475929042657754 ) ) ;
#38998=CARTESIAN_POINT ( 'NONE',  ( 35.45666904871060154, -273.7919793432992606, -289.0807834443223214 ) ) ;
#39000=CARTESIAN_POINT ( 'NONE',  ( -93.06368063729337337, -295.6687558741710973, -218.3082071701354607 ) ) ;
#39001=CARTESIAN_POINT ( 'NONE',  ( -106.7784570364784003, -291.8229331462158598, -295.3606620649267143 ) ) ;
#39002=CARTESIAN_POINT ( 'NONE',  ( -35.37928727901739734, -273.4259806303805931, -197.2730070036878658 ) ) ;
#39003=CARTESIAN_POINT ( 'NONE',  ( -105.7495009215837740, -291.7072954930050059, -297.9038311947999205 ) ) ;
#39004=CARTESIAN_POINT ( 'NONE',  ( -20.02812421946426724, -293.2212839492751755, -199.1493641275005757 ) ) ;
#39005=CARTESIAN_POINT ( 'NONE',  ( -106.1478100833931251, -285.9508422871128914, -297.7712611095400348 ) ) ;
#39006=CARTESIAN_POINT ( 'NONE',  ( -98.74203055571608445, -292.5869287079769947, -224.8572653843821456 ) ) ;
#39007=CARTESIAN_POINT ( 'NONE',  ( -19.51802461569899450, -293.5917902759066465, -195.9049372163300688 ) ) ;
#39008=CARTESIAN_POINT ( 'NONE',  ( -31.60447300687928163, -294.8111695704215549, -343.1854315091241006 ) ) ;
#39009=CARTESIAN_POINT ( 'NONE',  ( 17.49009224085631686, -290.2692810093295179, -321.6081756120736372 ) ) ;
#39010=CARTESIAN_POINT ( 'NONE',  ( 36.98445436032886136, -281.4663581058367754, -250.1958847455222781 ) ) ;
#39011=CARTESIAN_POINT ( 'NONE',  ( -106.9334094854790465, -271.0810729753886221, -240.2735777226524192 ) ) ;
#39012=CARTESIAN_POINT ( 'NONE',  ( -89.88469337680724891, -285.1683257312641331, -214.0015345207497717 ) ) ;
#39013=CARTESIAN_POINT ( 'NONE',  ( 33.67054222880698688, -277.8304909373571832, -293.3634708625016287 ) ) ;
#39014=CARTESIAN_POINT ( 'NONE',  ( -65.48205049319672355, -282.2233603389707355, -338.1630739897074704 ) ) ;
#39015=CARTESIAN_POINT ( 'NONE',  ( -4.345659689830434047, -284.4868507100807733, -202.9951867596554678 ) ) ;
#39016=CARTESIAN_POINT ( 'NONE',  ( -92.45207484672172882, -275.9696250686766348, -322.4282745601493048 ) ) ;
#39018=CARTESIAN_POINT ( 'NONE',  ( -97.58664566831039622, -283.4838571114924548, -311.7837312621551860 ) ) ;
#39019=CARTESIAN_POINT ( 'NONE',  ( -59.20357792795423535, -280.9803744199904258, -196.9440421983110525 ) ) ;
#39020=CARTESIAN_POINT ( 'NONE',  ( 38.06132436901835092, -286.4303283800328472, -255.9665318392303561 ) ) ;
#39021=CARTESIAN_POINT ( 'NONE',  ( -3.858454154786618684, -296.3644074586063653, -336.3817229864486080 ) ) ;
#39022=CARTESIAN_POINT ( 'NONE',  ( 9.007433788079975301, -276.2765173383014030, -209.8780773956021619 ) ) ;
#39024=CARTESIAN_POINT ( 'NONE',  ( 34.25432723298111171, -276.5239218767931675, -243.3924855000753382 ) ) ;
#39025=CARTESIAN_POINT ( 'NONE',  ( -56.60221595240335546, -277.1406179054495738, -340.8269144054496564 ) ) ;
#39027=CARTESIAN_POINT ( 'NONE',  ( -55.76915472440706623, -299.8146850906341001, -197.7784781163661876 ) ) ;
#39028=CARTESIAN_POINT ( 'NONE',  ( 35.17122925017660862, -285.3133092446726664, -251.8186930608801219 ) ) ;
#39029=CARTESIAN_POINT ( 'NONE',  ( -113.0165467630394431, -292.0339229065062909, -279.7263851790283411 ) ) ;
#39030=CARTESIAN_POINT ( 'NONE',  ( 23.60584574728441964, -291.9091297105313174, -229.6226505903001396 ) ) ;
#39032=CARTESIAN_POINT ( 'NONE',  ( -55.01336574191913797, -291.4852909817102500, -199.5105730226777325 ) ) ;
#39034=CARTESIAN_POINT ( 'NONE',  ( -100.4185050601238061, -291.0534040245203187, -313.9823191292185811 ) ) ;
#39035=CARTESIAN_POINT ( 'NONE',  ( -108.7080772574181822, -279.4128477741582515, -254.4692374015736220 ) ) ;
#39036=CARTESIAN_POINT ( 'NONE',  ( -51.72908787756697535, -296.7926990029499166, -194.9777508197268787 ) ) ;
#39037=CARTESIAN_POINT ( 'NONE',  ( 7.477779198380253511, -287.2968412953714505, -207.8093246656045210 ) ) ;
#39038=CARTESIAN_POINT ( 'NONE',  ( 0.2697523895151422435, -286.8721642800231280, -203.1811812881146295 ) ) ;
#39040=CARTESIAN_POINT ( 'NONE',  ( -104.6186879773106995, -285.2678979832265895, -241.8428550806414137 ) ) ;
#39041=CARTESIAN_POINT ( 'NONE',  ( 199.5529246190115202, 289.5492434123001999, -97.49731541809454427 ) ) ;
#39042=CARTESIAN_POINT ( 'NONE',  ( 178.2299433891311367, 253.8212103647281594, -165.6831904525195682 ) ) ;
#39043=CARTESIAN_POINT ( 'NONE',  ( 201.5605228849236994, 292.5236489450776389, -53.99999999998448175 ) ) ;
#39044=CARTESIAN_POINT ( 'NONE',  ( -43.23025606418143241, -276.3255762324919829, -343.2852335824551346 ) ) ;
#39045=CARTESIAN_POINT ( 'NONE',  ( -105.5604524385525878, -277.1150520375541646, -297.2019060886451030 ) ) ;
#39046=CARTESIAN_POINT ( 'NONE',  ( -88.01925875771564733, -273.0328617545135330, -212.3460600736322874 ) ) ;
#39047=CARTESIAN_POINT ( 'NONE',  ( -106.8307097481477967, -265.7384667639375380, -305.7804014683771925 ) ) ;
#39048=CARTESIAN_POINT ( 'NONE',  ( -103.1899387383158029, -276.7251046416644726, -309.4176808801952347 ) ) ;
#39049=CARTESIAN_POINT ( 'NONE',  ( -108.4888339475103862, -291.2642207992174122, -253.6910708394728999 ) ) ;
#39050=CARTESIAN_POINT ( 'NONE',  ( -82.88311288681744315, -298.2500014121351342, -208.4068894757872670 ) ) ;
#39051=CARTESIAN_POINT ( 'NONE',  ( -112.5436807083961099, -296.8410566850397458, -286.6150104496201152 ) ) ;
#39052=CARTESIAN_POINT ( 'NONE',  ( -41.03709630743936287, -295.2665969390627083, -343.2800913917124603 ) ) ;
#39054=CARTESIAN_POINT ( 'NONE',  ( -8.412901268750733408, -278.5965707293539708, -340.1779943506299446 ) ) ;
#39055=CARTESIAN_POINT ( 'NONE',  ( 38.80946278849148712, -281.1972177424339634, -281.3396101231168700 ) ) ;
#39056=CARTESIAN_POINT ( 'NONE',  ( -83.64357314639039487, -280.4794828301169787, -213.4591250477863582 ) ) ;
#39057=CARTESIAN_POINT ( 'NONE',  ( -39.90600557863260889, -278.8440571491466358, -346.3174016105907072 ) ) ;
#39058=CARTESIAN_POINT ( 'NONE',  ( -67.04062821060830402, -296.2297936189843313, -203.0171833125274645 ) ) ;
#39060=CARTESIAN_POINT ( 'NONE',  ( -101.8559310399065794, -278.2535160764398370, -304.5212411430550787 ) ) ;
#39061=CARTESIAN_POINT ( 'NONE',  ( -66.17613040871646035, -274.4870492672792466, -199.1238451561870590 ) ) ;
#39062=CARTESIAN_POINT ( 'NONE',  ( 37.02110170347383189, -286.4640280874083373, -288.4017372538645532 ) ) ;
#39063=CARTESIAN_POINT ( 'NONE',  ( -92.68705999424723530, -275.2592177793211476, -219.7270143720013778 ) ) ;
#39064=CARTESIAN_POINT ( 'NONE',  ( 0.7375189523886449550, -275.1298386140090884, -336.6674802013300791 ) ) ;
#39066=CARTESIAN_POINT ( 'NONE',  ( -105.2667651259092736, -289.3847149114924946, -297.6777755072259879 ) ) ;
#39067=CARTESIAN_POINT ( 'NONE',  ( -107.8293684223767315, -284.2946244181899829, -239.4903874724545005 ) ) ;
#39068=CARTESIAN_POINT ( 'NONE',  ( -8.114428241124437946, -280.9038493841821378, -338.3592105526763021 ) ) ;
#39069=CARTESIAN_POINT ( 'NONE',  ( 34.03148051693681708, -279.8916278831450200, -252.3865886998769668 ) ) ;
#39070=CARTESIAN_POINT ( 'NONE',  ( -107.8893236561030733, -282.9433505169986915, -246.4438844820208203 ) ) ;
#39071=CARTESIAN_POINT ( 'NONE',  ( -110.3029948668050508, -292.3286092238428182, -287.7833098781530907 ) ) ;
#39072=CARTESIAN_POINT ( 'NONE',  ( -43.80124609601869423, -281.1739228157629782, -197.1983356964263407 ) ) ;
#39073=CARTESIAN_POINT ( 'NONE',  ( 121.2562178857222364, 149.7689829628632197, -263.4557525892608965 ) ) ;
#39074=CARTESIAN_POINT ( 'NONE',  ( -83.41586613599116617, -282.0713700429554365, -331.1201782945501577 ) ) ;
#39075=CARTESIAN_POINT ( 'NONE',  ( 35.14292206396039830, -295.3041644955467291, -251.0507882953545504 ) ) ;
#39076=CARTESIAN_POINT ( 'NONE',  ( -105.2596579256097584, -277.2375362024735068, -236.1687128667616662 ) ) ;
#39077=CARTESIAN_POINT ( 'NONE',  ( -31.74671705337128103, -284.9818726723361806, -345.3322223354393827 ) ) ;
#39079=CARTESIAN_POINT ( 'NONE',  ( -61.25644552779765206, -293.6643020961961383, -198.6303524078388705 ) ) ;
#39080=CARTESIAN_POINT ( 'NONE',  ( -15.83096643689033911, -274.7738702360429670, -342.2646442902983495 ) ) ;
#39081=CARTESIAN_POINT ( 'NONE',  ( 23.73930902040109814, -286.1262571540097497, -223.7212068313149871 ) ) ;
#39082=CARTESIAN_POINT ( 'NONE',  ( -60.49078163218569415, -290.1468668022767474, -200.2321114891611842 ) ) ;
#39084=CARTESIAN_POINT ( 'NONE',  ( 12.06694098884280564, -275.0329944022522568, -324.8363142391011138 ) ) ;
#39085=CARTESIAN_POINT ( 'NONE',  ( 6.778348401442580773, -292.5847899992535304, -330.1268138434207913 ) ) ;
#39088=CARTESIAN_POINT ( 'NONE',  ( 37.38763089432415399, -292.2268243310051048, -285.7959759287206793 ) ) ;
#39089=CARTESIAN_POINT ( 'NONE',  ( -90.25045991324962813, -286.8888408193017767, -218.8377516844456636 ) ) ;
#39090=CARTESIAN_POINT ( 'NONE',  ( -43.12778944242869272, -287.3641256548171441, -346.1271736032116451 ) ) ;
#39091=CARTESIAN_POINT ( 'NONE',  ( 33.95495618862442910, -288.7381880323155769, -252.0850026225271563 ) ) ;
#39093=CARTESIAN_POINT ( 'NONE',  ( 32.47077699069772194, -288.6463593815438458, -292.4117572671948437 ) ) ;
#39094=CARTESIAN_POINT ( 'NONE',  ( 37.19344518559813650, -295.6737268671845413, -281.4479983466865178 ) ) ;
#39097=CARTESIAN_POINT ( 'NONE',  ( 26.02025418839926729, -288.1864000262094123, -227.2880529151445046 ) ) ;
#39098=CARTESIAN_POINT ( 'NONE',  ( -23.23223106991694209, -274.9530651570714213, -344.6452581387861756 ) ) ;
#39099=CARTESIAN_POINT ( 'NONE',  ( -114.0232400600147287, -278.9772664380271863, -263.0201646655798413 ) ) ;
#39100=CARTESIAN_POINT ( 'NONE',  ( -28.22329423508226043, -279.8314409507368055, -193.8706122946222195 ) ) ;
#39101=CARTESIAN_POINT ( 'NONE',  ( 10.21538519671316436, -300.6301984948891004, -195.7001660573785387 ) ) ;
#39103=CARTESIAN_POINT ( 'NONE',  ( -84.89686901255474538, -283.3965685805841304, -212.2979121390890498 ) ) ;
#39105=CARTESIAN_POINT ( 'NONE',  ( -109.9782047793844129, -276.4929592356365333, -285.6844229600759490 ) ) ;
#39106=CARTESIAN_POINT ( 'NONE',  ( 26.58656734916524300, -280.0792582632824974, -309.6790888600927474 ) ) ;
#39108=CARTESIAN_POINT ( 'NONE',  ( -51.20581444962512307, -275.7061765038387762, -345.3977362771613571 ) ) ;
#39110=CARTESIAN_POINT ( 'NONE',  ( -102.0671319982980805, -297.5958823943206539, -305.5935777317882298 ) ) ;
#39111=CARTESIAN_POINT ( 'NONE',  ( -31.67291075209326223, -281.9025378275022149, -346.8554240143182028 ) ) ;
#39112=CARTESIAN_POINT ( 'NONE',  ( -79.87440459920578917, -298.4020738051065678, -210.7425177149031867 ) ) ;
#39113=CARTESIAN_POINT ( 'NONE',  ( -99.53052609969535069, -298.4616263663543236, -225.7982612776796429 ) ) ;
#39114=CARTESIAN_POINT ( 'NONE',  ( -51.56142321081932778, -273.5320927703592702, -198.6860848071059138 ) ) ;
#39115=CARTESIAN_POINT ( 'NONE',  ( 23.41019998294785864, -294.9531667766371470, -226.3596651026312827 ) ) ;
#39116=CARTESIAN_POINT ( 'NONE',  ( 36.78498938113761341, -287.9805158355109143, -291.2477568069825224 ) ) ;
#39118=CARTESIAN_POINT ( 'NONE',  ( -68.06420618579394954, -277.7317965669738555, -201.3148241212551284 ) ) ;
#39119=CARTESIAN_POINT ( 'NONE',  ( -78.13820641377049014, -289.4175317387495738, -335.7275662592843446 ) ) ;
#39120=CARTESIAN_POINT ( 'NONE',  ( 22.14584001274747038, -287.2061345901546474, -313.0769349186299451 ) ) ;
#39121=CARTESIAN_POINT ( 'NONE',  ( 11.98281780226643534, -290.7376934790190148, -213.8625111247438895 ) ) ;
#39123=CARTESIAN_POINT ( 'NONE',  ( -49.37856652629597676, -155.6656457446864010, -366.7448178265262868 ) ) ;
#39124=CARTESIAN_POINT ( 'NONE',  ( -0.9662438810527488320, -288.0632857770915507, -333.7819143788195220 ) ) ;
#39126=CARTESIAN_POINT ( 'NONE',  ( -83.73144776340052431, -284.6123414491839299, -331.5900576903684396 ) ) ;
#39127=CARTESIAN_POINT ( 'NONE',  ( 4.024866690522677537, -291.6532025264916115, -205.6326011215083156 ) ) ;
#39128=CARTESIAN_POINT ( 'NONE',  ( 38.90978637575963717, -283.1466346999904999, -269.9144059094882664 ) ) ;
#39130=CARTESIAN_POINT ( 'NONE',  ( -25.48861644633841195, -281.5153657426774316, -194.7780333742352923 ) ) ;
#39131=CARTESIAN_POINT ( 'NONE',  ( 11.91512519495077704, -282.1777297027140889, -324.2384338361215441 ) ) ;
#39132=CARTESIAN_POINT ( 'NONE',  ( -114.3662121264988514, -296.5257802791869040, -272.4697928229329023 ) ) ;
#39133=CARTESIAN_POINT ( 'NONE',  ( -57.00959231293859375, -275.1084223918394400, -199.4954901923533725 ) ) ;
#39134=CARTESIAN_POINT ( 'NONE',  ( 7.688098436528640889, -290.6904391448102842, -210.8282359685273946 ) ) ;
#39135=CARTESIAN_POINT ( 'NONE',  ( -1.515474592538123444, -273.3332820062719293, -206.2872836043779330 ) ) ;
#39138=CARTESIAN_POINT ( 'NONE',  ( -110.0770768630098360, -286.6779795003275808, -254.4623533305098135 ) ) ;
#39139=CARTESIAN_POINT ( 'NONE',  ( 15.27663094474967664, -295.4091959345665259, -326.1536241480708895 ) ) ;
#39140=CARTESIAN_POINT ( 'NONE',  ( -104.6946986636557710, -285.5859788167392139, -241.8150223254299647 ) ) ;
#39141=CARTESIAN_POINT ( 'NONE',  ( -38.55330232588386252, -276.1257497584532530, -347.1162626573317311 ) ) ;
#39142=CARTESIAN_POINT ( 'NONE',  ( 23.02288617697955431, -293.5653158833952716, -222.7015498795072972 ) ) ;
#39143=CARTESIAN_POINT ( 'NONE',  ( 15.45568152725684463, -284.9286340258303767, -216.0219795157446185 ) ) ;
#39145=CARTESIAN_POINT ( 'NONE',  ( 22.19020729555418470, -293.2298965614671715, -221.5584921295464653 ) ) ;
#39146=CARTESIAN_POINT ( 'NONE',  ( -109.6432861772453862, -290.7493954880410456, -280.6766433401361382 ) ) ;
#39149=CARTESIAN_POINT ( 'NONE',  ( 202.6186562182569730, 291.9839156117442940, -53.99999999998471623 ) ) ;
#39150=CARTESIAN_POINT ( 'NONE',  ( -107.5812874519488958, -285.6877340002882306, -300.3141271305244118 ) ) ;
#39151=CARTESIAN_POINT ( 'NONE',  ( 25.18497378105905682, -273.6952119285918457, -320.2651865833026363 ) ) ;
#39153=CARTESIAN_POINT ( 'NONE',  ( -45.68825912565812786, -282.0806108211816650, -343.2447461898660208 ) ) ;
#39154=CARTESIAN_POINT ( 'NONE',  ( -114.2111188623227065, -278.1675406940815378, -274.4643794785486079 ) ) ;
#39155=CARTESIAN_POINT ( 'NONE',  ( -52.21607459267105611, -281.8615825287808434, -196.9679092636669395 ) ) ;
#39156=CARTESIAN_POINT ( 'NONE',  ( -101.4906385538783979, -256.4535248988104286, -325.6885106913075560 ) ) ;
#39157=CARTESIAN_POINT ( 'NONE',  ( -5.716086811928156486, -281.2190912455022271, -339.9199195617673013 ) ) ;
#39158=CARTESIAN_POINT ( 'NONE',  ( -19.39655578048297002, -284.3042442637076874, -197.9054860830946723 ) ) ;
#39159=CARTESIAN_POINT ( 'NONE',  ( -77.68371183542342351, -299.2785238985585465, -205.9678255979188464 ) ) ;
#39160=CARTESIAN_POINT ( 'NONE',  ( -47.79564887872264478, -295.6808908574199108, -342.7222144880499286 ) ) ;
#39161=ORIENTED_EDGE ( 'NONE', *, *, #26867, .F. ) ;
#39162=CARTESIAN_POINT ( 'NONE',  ( 33.10658487813985573, -291.9596945361947178, -249.2504135550059914 ) ) ;
#39163=CARTESIAN_POINT ( 'NONE',  ( -68.96586422155552043, -278.1085800970627133, -340.4699035502929405 ) ) ;
#39164=CARTESIAN_POINT ( 'NONE',  ( 0.6124664196134874672, -274.5735718893940316, -208.0034300710455568 ) ) ;
#39165=CARTESIAN_POINT ( 'NONE',  ( 39.07133972923853804, -274.5543815347095915, -276.8833759425634753 ) ) ;
#39167=CARTESIAN_POINT ( 'NONE',  ( 21.38441682075998784, -272.9106887342970253, -223.6906697486223834 ) ) ;
#39168=CARTESIAN_POINT ( 'NONE',  ( 1.485778912310653288, -295.9691076023856340, -336.1717034843913439 ) ) ;
#39172=CARTESIAN_POINT ( 'NONE',  ( -65.42143309300976739, -284.5077384583489675, -338.0929732961477612 ) ) ;
#39173=CARTESIAN_POINT ( 'NONE',  ( -16.39931441994946582, -284.5453960787947381, -343.4594389166588826 ) ) ;
#39174=CARTESIAN_POINT ( 'NONE',  ( -110.4924841550375305, -283.8936123408574304, -270.9017860693681996 ) ) ;
#39175=CARTESIAN_POINT ( 'NONE',  ( -13.54652497288685176, -275.1380186982442524, -340.2734753092330493 ) ) ;
#39176=CARTESIAN_POINT ( 'NONE',  ( -4.255718922491010581, -284.4716355098751137, -336.8154882768932907 ) ) ;
#39177=CARTESIAN_POINT ( 'NONE',  ( -39.19441413202154223, -275.5556986400789015, -344.0311607746497771 ) ) ;
#39178=CARTESIAN_POINT ( 'NONE',  ( 34.47012510449684441, -276.8254605182967225, -285.1018042379710096 ) ) ;
#39180=CARTESIAN_POINT ( 'NONE',  ( -114.2164696528975583, -279.3752018324797177, -268.7478607598796998 ) ) ;
#39181=CARTESIAN_POINT ( 'NONE',  ( -45.27326818481799364, -280.4467181314177537, -193.7796318452997468 ) ) ;
#39184=CARTESIAN_POINT ( 'NONE',  ( 32.70820596841620898, -289.0381642780544098, -241.3569490274842337 ) ) ;
#39185=CARTESIAN_POINT ( 'NONE',  ( -75.75151563270300414, -294.7759445622058365, -332.6880569481569410 ) ) ;
#39186=CARTESIAN_POINT ( 'NONE',  ( -62.73782756125602589, -288.7226680088817830, -343.0008268572557313 ) ) ;
#39187=CARTESIAN_POINT ( 'NONE',  ( -1.678702082059443157, -284.7710603968801024, -205.4489646690272764 ) ) ;
#39188=CARTESIAN_POINT ( 'NONE',  ( -14.36493683927242060, -284.9305665826997256, -200.3974148420774668 ) ) ;
#39189=CARTESIAN_POINT ( 'NONE',  ( -95.06734814741933803, -289.4379520340669956, -224.0190299883646219 ) ) ;
#39190=CARTESIAN_POINT ( 'NONE',  ( 4.941657197055613793, -287.8425488357234485, -210.3051975103153097 ) ) ;
#39191=CARTESIAN_POINT ( 'NONE',  ( -41.30491071720452823, -275.1018660214030547, -345.2692011847943832 ) ) ;
#39192=CARTESIAN_POINT ( 'NONE',  ( 35.18005549901627660, -286.2492492666621047, -293.7499053798907767 ) ) ;
#39193=CARTESIAN_POINT ( 'NONE',  ( -33.84668973151497795, -288.0962950621700429, -195.4425918820251411 ) ) ;
#39194=CARTESIAN_POINT ( 'NONE',  ( 31.18285516593091700, -285.9562495464727476, -301.2547054288272648 ) ) ;
#39195=CARTESIAN_POINT ( 'NONE',  ( -3.502037048887692627, -283.5352508045358491, -335.3234998129452720 ) ) ;
#39196=CARTESIAN_POINT ( 'NONE',  ( -95.84667634917079226, -291.9039756218037382, -317.5745879250472399 ) ) ;
#39199=CARTESIAN_POINT ( 'NONE',  ( -111.7259169901823697, -298.6415263055387186, -257.0832235117029541 ) ) ;
#39200=CARTESIAN_POINT ( 'NONE',  ( 28.60176447538386668, -280.0264956302277710, -306.0887000737391759 ) ) ;
#39201=CARTESIAN_POINT ( 'NONE',  ( 15.33492168232747588, -291.9706378633057966, -214.3476170998381463 ) ) ;
#39202=CARTESIAN_POINT ( 'NONE',  ( -110.1555178763190810, -294.7951160924662304, -282.3856080295178685 ) ) ;
#39203=CARTESIAN_POINT ( 'NONE',  ( 25.56702707961839494, -279.7163180401468594, -232.2659407596154324 ) ) ;
#39204=CARTESIAN_POINT ( 'NONE',  ( -63.79605198023946855, -271.7844004016682220, -200.7666052905431684 ) ) ;
#39205=CARTESIAN_POINT ( 'NONE',  ( -47.84708356565414533, -296.5035851753454494, -343.1511811434824040 ) ) ;
#39206=CARTESIAN_POINT ( 'NONE',  ( -34.06437162994986778, -296.5723644529182934, -194.0552759049878944 ) ) ;
#39207=CARTESIAN_POINT ( 'NONE',  ( 14.76727711359516704, -292.5698407363801152, -325.6659866909026277 ) ) ;
#39208=CARTESIAN_POINT ( 'NONE',  ( -36.21517100176666304, -293.4917875990831249, -196.7679327184013687 ) ) ;
#39210=CARTESIAN_POINT ( 'NONE',  ( 32.50399829062326518, -294.6429087089654786, -292.1367956863843460 ) ) ;
#39212=CARTESIAN_POINT ( 'NONE',  ( -24.83200130879724199, -280.9135769167810395, -344.7236589037539716 ) ) ;
#39213=CARTESIAN_POINT ( 'NONE',  ( -4.336659316753177507, -294.6045509917273648, -335.4878436705264448 ) ) ;
#39214=CARTESIAN_POINT ( 'NONE',  ( -69.18645551823109940, -283.4595737223696688, -340.4819622638265741 ) ) ;
#39215=CARTESIAN_POINT ( 'NONE',  ( -20.10885610051680672, -282.1919246494306890, -196.7387464819910292 ) ) ;
#39216=CARTESIAN_POINT ( 'NONE',  ( -91.88501575833059576, -284.9662400875823778, -216.0401182537028433 ) ) ;
#39217=CARTESIAN_POINT ( 'NONE',  ( -55.43148450691934670, -289.8186799472982216, -197.7471515260073431 ) ) ;
#39218=CARTESIAN_POINT ( 'NONE',  ( 29.14817507504886507, -280.5234630654710486, -307.9094349044098635 ) ) ;
#39219=CARTESIAN_POINT ( 'NONE',  ( 37.72379479509600486, -286.2744757424396198, -254.5919392249556665 ) ) ;
#39221=CARTESIAN_POINT ( 'NONE',  ( -92.77829237184437261, -297.4643602268567406, -319.0768716641624678 ) ) ;
#39222=CARTESIAN_POINT ( 'NONE',  ( 0.7690221592165564779, -277.9799232077851343, -336.6493755738805476 ) ) ;
#39223=CARTESIAN_POINT ( 'NONE',  ( 36.71359360977782416, -291.3941658529361689, -256.4248245494214871 ) ) ;
#39224=CARTESIAN_POINT ( 'NONE',  ( -66.07411270941601344, -279.3322056802392126, -203.2167376533870708 ) ) ;
#39225=CARTESIAN_POINT ( 'NONE',  ( -19.38883471001782155, -292.4434811104758865, -195.4284313988002566 ) ) ;
#39226=CARTESIAN_POINT ( 'NONE',  ( -66.60830445785840936, -283.7516311058159886, -200.6992197125136386 ) ) ;
#39227=CARTESIAN_POINT ( 'NONE',  ( -8.626191620539108484, -278.6765642235279188, -339.6600988359395501 ) ) ;
#39230=CARTESIAN_POINT ( 'NONE',  ( 19.87008729753278757, -293.2548619872140421, -316.1000268374112352 ) ) ;
#39231=CARTESIAN_POINT ( 'NONE',  ( -88.88668731264839096, -271.3304146053313275, -215.5804413312784789 ) ) ;
#39234=CARTESIAN_POINT ( 'NONE',  ( -38.34942626026715828, -294.5727733374662307, -343.4157066810456627 ) ) ;
#39236=CIRCLE ( 'NONE', #63501, 6.654241149514406040 ) ;
#39237=CARTESIAN_POINT ( 'NONE',  ( -102.0455923789670294, -287.6237833571632905, -301.4846348637937581 ) ) ;
#39238=CARTESIAN_POINT ( 'NONE',  ( -23.40085525011318879, -297.2814403089774942, -193.5985747488931565 ) ) ;
#39239=CARTESIAN_POINT ( 'NONE',  ( 13.90405535230756229, -288.0681059394203771, -213.4818634071896497 ) ) ;
#39240=CARTESIAN_POINT ( 'NONE',  ( 21.96045292213683098, -287.9805814045535612, -312.9317022882359538 ) ) ;
#39241=CARTESIAN_POINT ( 'NONE',  ( -109.8174618690418072, -280.2466066697485871, -257.0205140322607917 ) ) ;
#39242=CARTESIAN_POINT ( 'NONE',  ( -96.92929746259173385, -298.9193605371821718, -226.4387761807520008 ) ) ;
#39243=CARTESIAN_POINT ( 'NONE',  ( -27.48996652852445877, -278.9748759069121320, -197.5767535893036495 ) ) ;
#39245=CARTESIAN_POINT ( 'NONE',  ( -43.28388814980958443, -297.6459089744346329, -193.5587550616638168 ) ) ;
#39246=CARTESIAN_POINT ( 'NONE',  ( -14.42588679147071851, -294.2717350668584686, -199.5361245461241424 ) ) ;
#39247=CARTESIAN_POINT ( 'NONE',  ( 38.64179651915917191, -295.0797377589528310, -264.6210264208356762 ) ) ;
#39250=CARTESIAN_POINT ( 'NONE',  ( -110.3479786306968577, -291.2644785409744372, -265.7374262183761857 ) ) ;
#39252=CARTESIAN_POINT ( 'NONE',  ( -2.600766629777929051, -290.6461393623806657, -203.0162477819706908 ) ) ;
#39253=CARTESIAN_POINT ( 'NONE',  ( -68.05254770667625053, -297.3042076727552399, -204.0984398096427128 ) ) ;
#39256=CARTESIAN_POINT ( 'NONE',  ( -113.6757650018220289, -292.0971223824941490, -268.3920952787018450 ) ) ;
#39257=CARTESIAN_POINT ( 'NONE',  ( 25.22466315766300227, -290.6948066931273047, -320.2154176792147382 ) ) ;
#39258=CARTESIAN_POINT ( 'NONE',  ( -19.40037603436253733, -288.2836563974520914, -197.7103278067051804 ) ) ;
#39259=CARTESIAN_POINT ( 'NONE',  ( -5.731981148427274242, -272.4686196271861718, -202.5315219597227951 ) ) ;
#39260=CARTESIAN_POINT ( 'NONE',  ( 14.48196961711430575, -276.7083022451811303, -216.9231029507884330 ) ) ;
#39261=CARTESIAN_POINT ( 'NONE',  ( -80.34299539760660025, -289.5448267694019933, -209.5344511864218759 ) ) ;
#39262=CARTESIAN_POINT ( 'NONE',  ( -99.43932283705458985, -279.8293676274468567, -313.7683839085281647 ) ) ;
#39263=ORIENTED_EDGE ( 'NONE', *, *, #75203, .F. ) ;
#39264=CARTESIAN_POINT ( 'NONE',  ( -10.94669580006989484, -282.0474463661087725, -338.5851188835326866 ) ) ;
#39265=CARTESIAN_POINT ( 'NONE',  ( -108.3649693109729952, -279.2628577419237672, -299.2953147673320586 ) ) ;
#39266=CARTESIAN_POINT ( 'NONE',  ( 39.31318636514456699, -280.3418819737761396, -269.9478070697722387 ) ) ;
#39267=CARTESIAN_POINT ( 'NONE',  ( 197.4647849659431813, 287.3553758152445994, -96.51471344131978469 ) ) ;
#39268=CARTESIAN_POINT ( 'NONE',  ( 37.95392641538847300, -276.6808955572237778, -285.3073160645459438 ) ) ;
#39270=CARTESIAN_POINT ( 'NONE',  ( -69.85410986235015685, -275.1519190444135461, -201.3131386302572423 ) ) ;
#39271=CARTESIAN_POINT ( 'NONE',  ( 27.36219212280431989, -278.4805209788416391, -301.4846348637938149 ) ) ;
#39275=CARTESIAN_POINT ( 'NONE',  ( -72.49505816637696398, -290.6088331526117372, -334.6920397291250993 ) ) ;
#39276=CARTESIAN_POINT ( 'NONE',  ( -72.68242731066128215, -291.2736709485791380, -337.6438508129793377 ) ) ;
#39277=CARTESIAN_POINT ( 'NONE',  ( -109.8000173480027968, -290.0331828083702703, -260.3068860336741750 ) ) ;
#39278=CARTESIAN_POINT ( 'NONE',  ( -68.47010882348477878, -285.1616790808510586, -199.9866153932235875 ) ) ;
#39280=CARTESIAN_POINT ( 'NONE',  ( 22.44823254245317301, -280.5509465998648579, -313.6447904709196450 ) ) ;
#39281=CARTESIAN_POINT ( 'NONE',  ( -15.46541120563776417, -290.6265462162186850, -341.3535031152059105 ) ) ;
#39282=CARTESIAN_POINT ( 'NONE',  ( -70.54448389114365625, -281.9779698152066203, -336.1649177699672464 ) ) ;
#39283=CARTESIAN_POINT ( 'NONE',  ( 11.62199682767608344, -282.0640414943837868, -215.5541854168594398 ) ) ;
#39284=CARTESIAN_POINT ( 'NONE',  ( 19.45824493826854251, -289.1975058586792784, -322.0197022495066221 ) ) ;
#39285=CARTESIAN_POINT ( 'NONE',  ( -102.2134076509238554, -279.5025225748929074, -236.6407266879552367 ) ) ;
#39286=CARTESIAN_POINT ( 'NONE',  ( -113.6099547600766044, -289.4438718525689751, -262.6615319410354914 ) ) ;
#39287=CARTESIAN_POINT ( 'NONE',  ( -78.44473344933318515, -286.3166699123464696, -205.4404011655635429 ) ) ;
#39288=CARTESIAN_POINT ( 'NONE',  ( -36.57234973182783477, -286.5539098866731820, -193.4134744558207046 ) ) ;
#39289=CARTESIAN_POINT ( 'NONE',  ( -108.9790853781976381, -284.5336390521810586, -284.3998158941558927 ) ) ;
#39291=CARTESIAN_POINT ( 'NONE',  ( 144.2857639756989272, -299.5541904835127980, -189.2068768330456123 ) ) ;
#39292=CARTESIAN_POINT ( 'NONE',  ( -47.59998609859089669, -293.7836280128283306, -195.2410608317548792 ) ) ;
#39293=CARTESIAN_POINT ( 'NONE',  ( -11.24129318960841672, -293.4039942207975287, -342.3344044683004199 ) ) ;
#39294=CARTESIAN_POINT ( 'NONE',  ( 29.36366256375835704, -275.0170223632680404, -300.5902932201364592 ) ) ;
#39295=CARTESIAN_POINT ( 'NONE',  ( -30.60815077471541912, -294.3177082494300407, -346.9638078808094974 ) ) ;
#39297=CARTESIAN_POINT ( 'NONE',  ( -107.6574253200685547, -289.3220798146726906, -248.2640183937235179 ) ) ;
#39298=CARTESIAN_POINT ( 'NONE',  ( 17.82105747384601813, -292.4884735886940916, -319.7263859475435197 ) ) ;
#39299=CARTESIAN_POINT ( 'NONE',  ( -38.92142805470328426, -293.2369742287043550, -196.9810459899228476 ) ) ;
#39301=CARTESIAN_POINT ( 'NONE',  ( -14.40115280315599655, -290.3485889834909131, -198.7260271446300237 ) ) ;
#39303=CARTESIAN_POINT ( 'NONE',  ( 17.46314378952469326, -296.2697726892754986, -321.6357982095648254 ) ) ;
#39304=CARTESIAN_POINT ( 'NONE',  ( -21.06542623132290615, -289.7793954503864029, -341.7648388618358126 ) ) ;
#39305=CARTESIAN_POINT ( 'NONE',  ( -5.946555528809022384, -278.6214061465901750, -338.8647799437262051 ) ) ;
#39306=CARTESIAN_POINT ( 'NONE',  ( -94.92251092261561496, -276.6598835008269361, -320.8829840158118145 ) ) ;
#39307=CARTESIAN_POINT ( 'NONE',  ( -0.08755179755317563095, -273.8829805189726585, -203.0747441809488691 ) ) ;
#39308=CARTESIAN_POINT ( 'NONE',  ( 32.70139175005581933, -279.9629629010212852, -295.7181358301613159 ) ) ;
#39309=CARTESIAN_POINT ( 'NONE',  ( -39.95612857935881124, -275.4843307480408043, -346.5291870796427247 ) ) ;
#39310=CARTESIAN_POINT ( 'NONE',  ( -110.2230550656959736, -295.3659986220739597, -260.5141729916349504 ) ) ;
#39311=CARTESIAN_POINT ( 'NONE',  ( -103.9471565363187437, -275.0099693548993969, -235.7717892038255627 ) ) ;
#39312=CARTESIAN_POINT ( 'NONE',  ( -108.0408062550929316, -273.4509941876315224, -251.5785169547469309 ) ) ;
#39315=CARTESIAN_POINT ( 'NONE',  ( -51.40362738262570730, -287.2512183850509473, -344.3926585705142429 ) ) ;
#39316=CARTESIAN_POINT ( 'NONE',  ( 26.63754940813002037, -274.9040520871092212, -235.1038649520244519 ) ) ;
#39317=CARTESIAN_POINT ( 'NONE',  ( -23.31193716973744401, -288.8776533954240335, -346.1263001555414007 ) ) ;
#39318=CARTESIAN_POINT ( 'NONE',  ( -80.22584383435339817, -275.4735302329809770, -208.5649068823958032 ) ) ;
#39319=CARTESIAN_POINT ( 'NONE',  ( -106.6697043890098087, -294.1838755843298827, -298.5330232998869064 ) ) ;
#39320=CARTESIAN_POINT ( 'NONE',  ( -55.67358304561735594, -282.4794958268097389, -344.9808264294359219 ) ) ;
#39322=CARTESIAN_POINT ( 'NONE',  ( -111.2935469783898554, -276.7133963233690110, -257.7905639762915371 ) ) ;
#39324=CARTESIAN_POINT ( 'NONE',  ( -95.41922696600950360, -289.9755429035691350, -225.4820428757223283 ) ) ;
#39327=CARTESIAN_POINT ( 'NONE',  ( -37.53008654365596186, -290.0496729215050777, -195.3485651561823033 ) ) ;
#39328=CARTESIAN_POINT ( 'NONE',  ( -31.30200224120455843, -275.6499083600147628, -196.9029277449011488 ) ) ;
#39329=CARTESIAN_POINT ( 'NONE',  ( -24.61372194124369273, -284.3181932555432354, -345.7580688073879287 ) ) ;
#39330=CARTESIAN_POINT ( 'NONE',  ( 24.16914792535496659, -273.0394208769029660, -226.4558368042394818 ) ) ;
#39331=CARTESIAN_POINT ( 'NONE',  ( -90.74146049882578779, -283.8363703792340402, -320.1352638049352208 ) ) ;
#39332=CARTESIAN_POINT ( 'NONE',  ( -21.82736098460249607, -275.6801792865140328, -198.4258679561123699 ) ) ;
#39333=CARTESIAN_POINT ( 'NONE',  ( -5.246425846308414798, -275.2885298001637580, -204.6015794358588948 ) ) ;
#39334=CARTESIAN_POINT ( 'NONE',  ( -31.75906638102517121, -284.9818726717181221, -345.1659850968312639 ) ) ;
#39335=ADVANCED_FACE ( 'NONE', ( #57205 ), #2172, .F. ) ;
#39337=CARTESIAN_POINT ( 'NONE',  ( 203.9781100709074906, 292.2290856633177327, -53.99999999998790656 ) ) ;
#39338=CARTESIAN_POINT ( 'NONE',  ( 29.57361841262769886, -293.8814194832198723, -308.5652814451379982 ) ) ;
#39339=CARTESIAN_POINT ( 'NONE',  ( -60.51260985763347833, -287.7300306075464960, -199.4036959377695837 ) ) ;
#39341=CARTESIAN_POINT ( 'NONE',  ( -119.3990491898856732, -288.0523547857347353, -270.3284710469131937 ) ) ;
#39342=CARTESIAN_POINT ( 'NONE',  ( -112.0206741183781531, -277.5219310159710631, -288.5051951738792582 ) ) ;
#39343=CARTESIAN_POINT ( 'NONE',  ( -76.73802342891927708, -289.9343341773857787, -205.0747402354498945 ) ) ;
#39344=CARTESIAN_POINT ( 'NONE',  ( -97.14874021825423256, -286.6689279724830612, -227.2835070044734209 ) ) ;
#39345=CARTESIAN_POINT ( 'NONE',  ( -7.073009339664039885, -278.4096030137305320, -337.9020712899364867 ) ) ;
#39346=CARTESIAN_POINT ( 'NONE',  ( 2.418795387446579959, -287.9993242518474972, -205.1099931741326827 ) ) ;
#39347=CARTESIAN_POINT ( 'NONE',  ( -31.97792536911539685, -284.9846209709714344, -345.1690759134061750 ) ) ;
#39348=CARTESIAN_POINT ( 'NONE',  ( -48.49188936316339493, -277.3568926635672369, -346.6034186737189202 ) ) ;
#39349=CARTESIAN_POINT ( 'NONE',  ( -54.13331621003629124, -277.0952148529740384, -345.5625591572148778 ) ) ;
#39350=CARTESIAN_POINT ( 'NONE',  ( -111.8154482312025237, -298.4934762073689285, -268.7251782247659548 ) ) ;
#39355=CARTESIAN_POINT ( 'NONE',  ( 7.109802698612255334, -296.7425731821555814, -194.6102166994000982 ) ) ;
#39357=CARTESIAN_POINT ( 'NONE',  ( -70.48631613441757793, -277.0091378617260034, -335.4719686269543217 ) ) ;
#39358=CARTESIAN_POINT ( 'NONE',  ( -18.66173394645513639, -275.4924843028174450, -196.0159471884904292 ) ) ;
#39360=CARTESIAN_POINT ( 'NONE',  ( 37.91250760616882332, -280.8009992371690942, -285.5144817020773758 ) ) ;
#39361=CARTESIAN_POINT ( 'NONE',  ( -16.91340317285666472, -288.0795991765610324, -199.1692346478915852 ) ) ;
#39362=CARTESIAN_POINT ( 'NONE',  ( -108.7815380698851868, -297.7282887020181761, -297.3253355459070804 ) ) ;
#39363=CARTESIAN_POINT ( 'NONE',  ( -93.38843113568697163, -297.0414993757552793, -322.5989414986647716 ) ) ;
#39364=CARTESIAN_POINT ( 'NONE',  ( -55.48079342112846746, -293.8183571034266492, -197.7594532776019776 ) ) ;
#39365=CARTESIAN_POINT ( 'NONE',  ( -34.21177587356489624, -278.0914102176075744, -195.5804055599008393 ) ) ;
#39366=CARTESIAN_POINT ( 'NONE',  ( 34.11005880877600305, -283.2014305034372228, -249.4814545779736363 ) ) ;
#39367=CARTESIAN_POINT ( 'NONE',  ( -107.8520031293320471, -270.8908921432557690, -245.8632819064056321 ) ) ;
#39368=CARTESIAN_POINT ( 'NONE',  ( -113.5408757646612656, -286.1567666718097485, -270.0060888298507962 ) ) ;
#39369=CARTESIAN_POINT ( 'NONE',  ( 35.96415068357816835, -286.4815592327109357, -271.0527171521861192 ) ) ;
#39370=CARTESIAN_POINT ( 'NONE',  ( 38.32378069700226320, -281.0733851889031030, -284.1472664677301623 ) ) ;
#39371=CARTESIAN_POINT ( 'NONE',  ( 104.8672404336123662, 115.1756038169428820, -282.3939451955034201 ) ) ;
#39372=ORIENTED_EDGE ( 'NONE', *, *, #20462, .T. ) ;
#39373=CARTESIAN_POINT ( 'NONE',  ( 23.55404352819028446, -286.6588602852423264, -229.9732141583376972 ) ) ;
#39375=CARTESIAN_POINT ( 'NONE',  ( -111.1900897473225882, -285.3715620525608756, -291.0470518728193952 ) ) ;
#39376=CARTESIAN_POINT ( 'NONE',  ( 22.48559948038277057, -276.4701542840274442, -312.3141692455732255 ) ) ;
#39377=CARTESIAN_POINT ( 'NONE',  ( 0.1031674301827133072, -285.3340557518053515, -203.5188271791187731 ) ) ;
#39379=CARTESIAN_POINT ( 'NONE',  ( -96.33225375960206804, -290.1343310065495871, -221.3346342840754062 ) ) ;
#39380=CARTESIAN_POINT ( 'NONE',  ( 19.94508063452825652, -281.7982973283400838, -219.2429714974994681 ) ) ;
#39382=CARTESIAN_POINT ( 'NONE',  ( -90.58835705372274560, -280.8346987716189460, -215.6293970588049831 ) ) ;
#39383=CARTESIAN_POINT ( 'NONE',  ( 37.84579318765830180, -282.0927320991972351, -286.9321597870633127 ) ) ;
#39384=CARTESIAN_POINT ( 'NONE',  ( -92.08974858914540107, -281.4094976428775112, -313.9805196606274080 ) ) ;
#39385=CARTESIAN_POINT ( 'NONE',  ( -83.35433501583091243, -219.9715334812069614, -352.6155196686340787 ) ) ;
#39386=ORIENTED_EDGE ( 'NONE', *, *, #75203, .T. ) ;
#39387=CARTESIAN_POINT ( 'NONE',  ( 35.96552309920986090, -277.7458007094012373, -285.3970566872844188 ) ) ;
#39388=CARTESIAN_POINT ( 'NONE',  ( -84.73245238795870193, -218.9744008934607677, -352.0618779874953930 ) ) ;
#39389=CARTESIAN_POINT ( 'NONE',  ( 16.46206323133144878, -278.8410301536602560, -218.5474991839913343 ) ) ;
#39390=CARTESIAN_POINT ( 'NONE',  ( -47.27840444084209537, -297.2712796092406506, -197.8863971304570839 ) ) ;
#39391=CARTESIAN_POINT ( 'NONE',  ( -92.76339991600542589, -290.7916625009636959, -216.9190290128747733 ) ) ;
#39393=CARTESIAN_POINT ( 'NONE',  ( -113.8479272357090224, -271.2730514282568492, -267.4953093779189999 ) ) ;
#39394=CARTESIAN_POINT ( 'NONE',  ( 33.44300810395984058, -285.6782063436313024, -249.4367087552971896 ) ) ;
#39395=CARTESIAN_POINT ( 'NONE',  ( 32.96332416060278803, -295.0992764220783329, -246.3670528101350783 ) ) ;
#39396=CARTESIAN_POINT ( 'NONE',  ( -19.71367887470570679, -287.5987801801365435, -199.0134036303937535 ) ) ;
#39398=CARTESIAN_POINT ( 'NONE',  ( 29.26551624276460828, -293.9960542012869382, -232.1996329519579660 ) ) ;
#39399=CARTESIAN_POINT ( 'NONE',  ( -90.78219977634950055, -284.3286381202823350, -320.1818108625622585 ) ) ;
#39400=CARTESIAN_POINT ( 'NONE',  ( -114.0320774532610812, -271.5085161411282684, -267.4914475766567534 ) ) ;
#39401=CARTESIAN_POINT ( 'NONE',  ( -50.54867280931357953, -292.6904255554932206, -194.6661069670267352 ) ) ;
#39402=CARTESIAN_POINT ( 'NONE',  ( -108.3127885092914369, -291.4226761038412974, -240.6520029324727830 ) ) ;
#39403=CARTESIAN_POINT ( 'NONE',  ( 3.616363193716710445, -288.6510550656896612, -330.8491941804259113 ) ) ;
#39406=CARTESIAN_POINT ( 'NONE',  ( -88.78725214128012055, -299.1998239713085468, -214.6693415879454960 ) ) ;
#39407=CARTESIAN_POINT ( 'NONE',  ( -112.6749436771190602, -271.5252420894163379, -256.1889733280397650 ) ) ;
#39408=CARTESIAN_POINT ( 'NONE',  ( 34.71480816512652723, -280.7839039600362412, -283.5182673523386256 ) ) ;
#39410=ORIENTED_EDGE ( 'NONE', *, *, #48459, .T. ) ;
#39411=CARTESIAN_POINT ( 'NONE',  ( -48.49127145023283703, -276.6979715578750643, -346.5412725406817458 ) ) ;
#39412=CARTESIAN_POINT ( 'NONE',  ( -99.01732784681938426, -295.5868639402693816, -229.9348940629868423 ) ) ;
#39413=CARTESIAN_POINT ( 'NONE',  ( -89.94464095535288095, -279.6646816932357638, -322.8153463981730056 ) ) ;
#39414=CARTESIAN_POINT ( 'NONE',  ( -21.65022116096443838, -272.3950198152109010, -197.8032585511467971 ) ) ;
#39415=CARTESIAN_POINT ( 'NONE',  ( -44.62366856959528860, -299.1631778943439031, -197.2755151012489137 ) ) ;
#39416=CARTESIAN_POINT ( 'NONE',  ( -109.5828009065488402, -297.7956066439823530, -257.8931818092237904 ) ) ;
#39417=CARTESIAN_POINT ( 'NONE',  ( -113.5382024664509402, -298.1615101387588425, -269.6307449282184621 ) ) ;
#39418=CARTESIAN_POINT ( 'NONE',  ( -77.93385925765447553, -271.5296901496937494, -206.8734544676563871 ) ) ;
#39419=CARTESIAN_POINT ( 'NONE',  ( 34.42602821600245733, -294.3867119136889983, -284.2638456570648486 ) ) ;
#39420=CARTESIAN_POINT ( 'NONE',  ( -32.09732282844340290, -290.6942902907457551, -196.9462744039742859 ) ) ;
#39422=CARTESIAN_POINT ( 'NONE',  ( -2.590953013314785114, -274.9916180478309116, -201.7030557405360867 ) ) ;
#39423=CARTESIAN_POINT ( 'NONE',  ( -35.81928768007912112, -298.4050094559723334, -197.3398847052345388 ) ) ;
#39424=CARTESIAN_POINT ( 'NONE',  ( -85.80301146869595641, -282.3921359563429405, -329.5624657254462591 ) ) ;
#39426=CARTESIAN_POINT ( 'NONE',  ( -45.66797648873498616, -282.3574050291476851, -343.0983647735912427 ) ) ;
#39427=CARTESIAN_POINT ( 'NONE',  ( -111.3369149988693465, -282.3789735844816278, -283.8662294229106919 ) ) ;
#39428=ADVANCED_FACE ( 'NONE', ( #36333 ), #55094, .F. ) ;
#39429=CARTESIAN_POINT ( 'NONE',  ( 18.74582431062491850, -274.7988787307726284, -318.0010646748665977 ) ) ;
#39430=CARTESIAN_POINT ( 'NONE',  ( 32.35641970274551937, -283.9146217680333848, -298.1977297619083629 ) ) ;
#39433=CARTESIAN_POINT ( 'NONE',  ( -35.52224807768872239, -272.4744712586767150, -194.1698466212318408 ) ) ;
#39434=CARTESIAN_POINT ( 'NONE',  ( -108.8145862638233581, -280.8541387049481841, -246.9222601696184825 ) ) ;
#39436=CARTESIAN_POINT ( 'NONE',  ( -71.07352685953270566, -285.4140054913966082, -337.9738243863387765 ) ) ;
#39438=CARTESIAN_POINT ( 'NONE',  ( -86.29322184692237840, -287.7308180053328215, -327.2508025193205299 ) ) ;
#39440=CARTESIAN_POINT ( 'NONE',  ( -90.70643078340208376, -294.6245137195579105, -320.8261543529608844 ) ) ;
#39441=CARTESIAN_POINT ( 'NONE',  ( -40.02613873826641822, -287.2256944840024744, -344.5981888845363983 ) ) ;
#39442=CARTESIAN_POINT ( 'NONE',  ( -94.07136297056315755, -227.2831051785662737, -345.8935872616412439 ) ) ;
#39443=CARTESIAN_POINT ( 'NONE',  ( -112.2402595566569801, -294.5019180862730082, -274.2606617501634219 ) ) ;
#39444=CARTESIAN_POINT ( 'NONE',  ( -101.9213024232333140, -283.5691575445194417, -229.7140674216624916 ) ) ;
#39445=CARTESIAN_POINT ( 'NONE',  ( -1.596244285866922130, -282.1345257086524043, -205.7956256302265672 ) ) ;
#39446=CARTESIAN_POINT ( 'NONE',  ( -0.8816117824729906571, -280.8148015125112238, -337.0439616038644317 ) ) ;
#39447=CARTESIAN_POINT ( 'NONE',  ( -31.87135465118553412, -288.9813445993796108, -343.2064891216612068 ) ) ;
#39448=CARTESIAN_POINT ( 'NONE',  ( 34.33017151230868791, -282.7590313300437401, -253.6722673727451820 ) ) ;
#39449=CARTESIAN_POINT ( 'NONE',  ( 34.72438982383177830, -282.1889724468341569, -257.7484098556087133 ) ) ;
#39450=CARTESIAN_POINT ( 'NONE',  ( 20.80456886803262861, -288.8739467082240822, -222.4297273436147577 ) ) ;
#39451=CARTESIAN_POINT ( 'NONE',  ( -29.06176134435187564, -298.3198158566332836, -193.3608907624496283 ) ) ;
#39453=CARTESIAN_POINT ( 'NONE',  ( -93.17216557534000287, -273.2770318234245224, -217.3139676789490409 ) ) ;
#39454=CARTESIAN_POINT ( 'NONE',  ( 20.60709865574768784, -294.8807720032332327, -223.2900503420511598 ) ) ;
#39456=CARTESIAN_POINT ( 'NONE',  ( -20.19161114001083490, -279.3376638359844719, -345.3538533559490702 ) ) ;
#39458=CARTESIAN_POINT ( 'NONE',  ( 22.05334534205814734, -274.1823983539516689, -316.4499450874267836 ) ) ;
#39460=CARTESIAN_POINT ( 'NONE',  ( -113.1494281489257503, -294.8544379786490595, -278.0830857777785923 ) ) ;
#39461=CARTESIAN_POINT ( 'NONE',  ( -36.72689055191467133, -273.4086625487323090, -197.2493374621504358 ) ) ;
#39462=CARTESIAN_POINT ( 'NONE',  ( -108.4257412633100301, -292.3266485621357447, -250.9248927945805860 ) ) ;
#39463=CARTESIAN_POINT ( 'NONE',  ( 20.15320880504508239, -283.9628890537467214, -316.9891425258840059 ) ) ;
#39464=CARTESIAN_POINT ( 'NONE',  ( -81.60394424953923931, -292.8878585811157791, -208.0758064170695150 ) ) ;
#39465=CARTESIAN_POINT ( 'NONE',  ( -99.63928747872814995, -292.4593067683714480, -225.9504336414273098 ) ) ;
#39466=CARTESIAN_POINT ( 'NONE',  ( 35.64185255868094515, -293.4267605252102271, -273.4910876524156720 ) ) ;
#39467=CARTESIAN_POINT ( 'NONE',  ( 28.80610798149704621, -290.0225726947860494, -305.8195370953117731 ) ) ;
#39468=CARTESIAN_POINT ( 'NONE',  ( 33.56675751606402969, -282.1023878138273631, -300.5137983929928964 ) ) ;
#39469=CARTESIAN_POINT ( 'NONE',  ( -98.73696105212438567, -295.2268209213725072, -226.3164118804131135 ) ) ;
#39470=CARTESIAN_POINT ( 'NONE',  ( -33.06086875028397998, -282.8329825812398894, -347.2551640514894871 ) ) ;
#39471=CARTESIAN_POINT ( 'NONE',  ( 35.19065165195718947, -277.7601887854273173, -288.0475296649000825 ) ) ;
#39472=CARTESIAN_POINT ( 'NONE',  ( -74.74732862405285516, -275.6841686836183385, -336.2483279547302004 ) ) ;
#39474=CARTESIAN_POINT ( 'NONE',  ( -38.89266775796220088, -282.5797451354689542, -343.4186940332111249 ) ) ;
#39475=CARTESIAN_POINT ( 'NONE',  ( -68.52501057723200972, -280.8565210478287213, -200.3781700284350791 ) ) ;
#39476=CARTESIAN_POINT ( 'NONE',  ( 18.46550512483153028, -287.3329708841433785, -323.0714211002008938 ) ) ;
#39477=CARTESIAN_POINT ( 'NONE',  ( 20.11850829645359084, -294.6610565969639310, -223.6902672264335763 ) ) ;
#39478=CARTESIAN_POINT ( 'NONE',  ( 21.12999181155816331, -277.8166928310874937, -319.2231856773271375 ) ) ;
#39479=CARTESIAN_POINT ( 'NONE',  ( 39.13744086591733407, -276.8414087900904406, -268.3021706118074121 ) ) ;
#39480=CARTESIAN_POINT ( 'NONE',  ( -90.96929360578974411, -277.6734542073776311, -319.9632383244808125 ) ) ;
#39481=CARTESIAN_POINT ( 'NONE',  ( -72.54952591492519787, -299.5851584090474944, -204.3129529917309810 ) ) ;
#39482=CARTESIAN_POINT ( 'NONE',  ( -3.749311614363324718, -284.4963017828312104, -203.4912453617877190 ) ) ;
#39483=CARTESIAN_POINT ( 'NONE',  ( 4.212312833704223713, -294.1755038163753966, -335.2236302310901692 ) ) ;
#39484=CARTESIAN_POINT ( 'NONE',  ( -57.06398587337482553, -290.9024232745837821, -344.0191233604846843 ) ) ;
#39486=CARTESIAN_POINT ( 'NONE',  ( 35.60436343034251649, -292.3702979548440908, -262.5827232592980636 ) ) ;
#39487=CARTESIAN_POINT ( 'NONE',  ( 14.89360017505270228, -292.4801586074845545, -219.2635910995844313 ) ) ;
#39489=CARTESIAN_POINT ( 'NONE',  ( -103.5246886435165692, -291.1242876625852887, -309.2127964404897966 ) ) ;
#39490=CARTESIAN_POINT ( 'NONE',  ( -107.3271000201876006, -279.4827603638244113, -249.2439100650014154 ) ) ;
#39491=EDGE_CURVE ( 'NONE', #64985, #9910, #9729, .T. ) ;
#39492=CARTESIAN_POINT ( 'NONE',  ( -112.3059315314913249, -295.2692924983359717, -286.5430993583566419 ) ) ;
#39493=CARTESIAN_POINT ( 'NONE',  ( -99.26709784780788937, -285.8110466102579039, -224.6822880096740391 ) ) ;
#39494=CARTESIAN_POINT ( 'NONE',  ( 39.55626317759415400, -287.8285666947950290, -265.8154133698561736 ) ) ;
#39495=CARTESIAN_POINT ( 'NONE',  ( -109.4426836976394384, -285.0388752939804249, -258.7261244418466504 ) ) ;
#39496=CARTESIAN_POINT ( 'NONE',  ( -78.32199257514537294, -208.3160289897915618, -357.0357957823952688 ) ) ;
#39497=CARTESIAN_POINT ( 'NONE',  ( 183.6448409953721068, 263.3645142227682641, -152.5370271569391605 ) ) ;
#39498=CARTESIAN_POINT ( 'NONE',  ( 200.3489741029065101, 290.3571495942200613, -82.34907451253036470 ) ) ;
#39500=CARTESIAN_POINT ( 'NONE',  ( -97.78799147175118378, -277.1771591182297811, -311.5781968440978176 ) ) ;
#39501=CARTESIAN_POINT ( 'NONE',  ( -43.24563289694334856, -276.0487820814591373, -343.4321084754016624 ) ) ;
#39502=CARTESIAN_POINT ( 'NONE',  ( -73.24632235394444990, -297.0970792890462349, -202.2553899741700150 ) ) ;
#39503=CARTESIAN_POINT ( 'NONE',  ( 186.0019925103573826, 260.3827756688246495, -151.4387398898385300 ) ) ;
#39504=CARTESIAN_POINT ( 'NONE',  ( -73.87618826675560513, -276.2117220566859714, -337.5960332078474266 ) ) ;
#39505=CARTESIAN_POINT ( 'NONE',  ( -29.91010277892296543, -275.9076503794852897, -196.7218256594801460 ) ) ;
#39506=CARTESIAN_POINT ( 'NONE',  ( -96.60486256646255754, -290.4474137011943640, -313.0912714994801149 ) ) ;
#39507=CARTESIAN_POINT ( 'NONE',  ( -93.55162380140724565, -298.0713291434958023, -217.8945343081029478 ) ) ;
#39508=CARTESIAN_POINT ( 'NONE',  ( -99.87519521369294750, -297.6389324643556051, -225.5382566759741962 ) ) ;
#39509=CARTESIAN_POINT ( 'NONE',  ( -69.72216010194318869, -295.6575341551252905, -335.7866926183041869 ) ) ;
#39511=CARTESIAN_POINT ( 'NONE',  ( 5.083347969299850000, -278.4035571443839672, -332.8865487279412037 ) ) ;
#39512=CARTESIAN_POINT ( 'NONE',  ( -18.93919614269879048, -282.3291811168978711, -345.1212832107209465 ) ) ;
#39513=CARTESIAN_POINT ( 'NONE',  ( -53.99582515532129179, -278.2123704211160771, -341.7299628314298161 ) ) ;
#39514=CARTESIAN_POINT ( 'NONE',  ( 35.10338877093467147, -277.6043020401518788, -293.2888982509517177 ) ) ;
#39515=CARTESIAN_POINT ( 'NONE',  ( -40.52544210569926975, -296.5860943348123442, -196.8281392923204578 ) ) ;
#39517=CARTESIAN_POINT ( 'NONE',  ( -91.29824953101562812, -279.4239033647737074, -221.1910988546306100 ) ) ;
#39518=CARTESIAN_POINT ( 'NONE',  ( -1.386125550053831201, -275.3195223355920120, -202.4541560592924156 ) ) ;
#39519=CARTESIAN_POINT ( 'NONE',  ( 38.18538596417830178, -286.3946528426932900, -282.8875900945142803 ) ) ;
#39520=CARTESIAN_POINT ( 'NONE',  ( -24.52705601584984052, -276.2157303281430245, -196.4112334349327114 ) ) ;
#39521=CARTESIAN_POINT ( 'NONE',  ( 31.31779611622292236, -274.5621408734106694, -304.0148409389797166 ) ) ;
#39523=CARTESIAN_POINT ( 'NONE',  ( -82.65426739764424724, -288.8870834772864100, -327.8012866266201968 ) ) ;
#39524=CARTESIAN_POINT ( 'NONE',  ( -112.1219757187193409, -283.6755994814863016, -288.3395832999151480 ) ) ;
#39525=CARTESIAN_POINT ( 'NONE',  ( 24.97164517709344622, -280.3380760612016616, -310.3930068161527629 ) ) ;
#39526=CARTESIAN_POINT ( 'NONE',  ( 33.68704139694921196, -279.8741471083410488, -251.0698688757379102 ) ) ;
#39527=CARTESIAN_POINT ( 'NONE',  ( -111.4250203434557704, -282.7327101095763737, -262.5756090973935670 ) ) ;
#39528=CARTESIAN_POINT ( 'NONE',  ( 20.26165323421227882, -290.2158563739235433, -318.4105624031598154 ) ) ;
#39529=CARTESIAN_POINT ( 'NONE',  ( -94.75408410926364411, -279.1147150926993277, -316.1080809135002028 ) ) ;
#39531=CARTESIAN_POINT ( 'NONE',  ( 35.70586767038074072, -280.2290987185073163, -292.2333273351335379 ) ) ;
#39532=CARTESIAN_POINT ( 'NONE',  ( -14.36976991830608519, -296.7544549676699148, -341.7564334400602206 ) ) ;
#39533=CARTESIAN_POINT ( 'NONE',  ( -36.73779531599069514, -278.2995094804257405, -194.3639735198903225 ) ) ;
#39534=CARTESIAN_POINT ( 'NONE',  ( -36.45662826106128307, -277.6922210603075882, -343.4701778058862374 ) ) ;
#39535=CARTESIAN_POINT ( 'NONE',  ( -64.56390392834998693, -285.4068306245200120, -340.4390952921592088 ) ) ;
#39538=DIRECTION ( 'NONE',  ( 1.000000000000000000, 0.000000000000000000, 0.000000000000000000 ) ) ;
#39539=CARTESIAN_POINT ( 'NONE',  ( -110.6044890883900962, -292.7086618137713003, -251.8189914200655721 ) ) ;
#39540=CARTESIAN_POINT ( 'NONE',  ( 39.19480708611742159, -286.6568534857642589, -262.9829575811123732 ) ) ;
#39541=CARTESIAN_POINT ( 'NONE',  ( -44.35617560996669084, -290.3619624410597453, -196.8438500617731961 ) ) ;
#39543=CARTESIAN_POINT ( 'NONE',  ( 3.393623833971007198, -275.1765498547301831, -331.5320004258667836 ) ) ;
#39544=CARTESIAN_POINT ( 'NONE',  ( 22.30503788460377024, -292.3011106193121122, -314.5553724384204202 ) ) ;
#39546=CARTESIAN_POINT ( 'NONE',  ( 38.16870806871002486, -291.8887970428065159, -259.0111584744097399 ) ) ;
#39547=CARTESIAN_POINT ( 'NONE',  ( -110.2142911208002687, -286.3055179672390977, -258.6179202281561516 ) ) ;
#39548=CARTESIAN_POINT ( 'NONE',  ( 17.89263496086532257, -286.5142137692236588, -322.5448533879898037 ) ) ;
#39549=CARTESIAN_POINT ( 'NONE',  ( -33.22369036685279298, -287.5301557072505148, -196.8369752689445704 ) ) ;
#39551=CARTESIAN_POINT ( 'NONE',  ( 35.43397495977787770, -288.2562236379149567, -262.8575959919190268 ) ) ;
#39552=CARTESIAN_POINT ( 'NONE',  ( -9.150464633899238365, -294.3988370069307052, -200.4779222555517038 ) ) ;
#39553=CARTESIAN_POINT ( 'NONE',  ( -74.64693530627204154, -275.6244402020410575, -336.0698208081736311 ) ) ;
#39555=CARTESIAN_POINT ( 'NONE',  ( -111.8059065654491349, -278.6405037740643138, -289.9276711227866485 ) ) ;
#39556=CARTESIAN_POINT ( 'NONE',  ( 34.09927956404828819, -291.3141040677170963, -245.5956636797952513 ) ) ;
#39557=CARTESIAN_POINT ( 'NONE',  ( -111.7310279967723403, -278.8016461197647686, -250.4298744472197598 ) ) ;
#39558=CARTESIAN_POINT ( 'NONE',  ( -108.2775947103428535, -298.8355497049901146, -246.9603479777366886 ) ) ;
#39560=CARTESIAN_POINT ( 'NONE',  ( -111.9822501674346142, -282.6527165842720137, -262.5162098752384168 ) ) ;
#39562=CARTESIAN_POINT ( 'NONE',  ( -110.5074648862690907, -276.5278871823754798, -282.9917234980234184 ) ) ;
#39563=CARTESIAN_POINT ( 'NONE',  ( 20.06237325652579884, -280.2192876587023420, -318.6288402295327273 ) ) ;
#39565=CARTESIAN_POINT ( 'NONE',  ( 23.80040341266763804, -274.6449210392831901, -316.0158102821628177 ) ) ;
#39567=CARTESIAN_POINT ( 'NONE',  ( -68.79585177553632036, -296.9933984051726270, -337.0183883640967224 ) ) ;
#39568=CARTESIAN_POINT ( 'NONE',  ( -0.5359154468656786019, -281.4951614167088110, -337.6576926782354349 ) ) ;
#39569=CARTESIAN_POINT ( 'NONE',  ( -102.7478552766864226, -297.9404755921403876, -237.3021005556155671 ) ) ;
#39570=CARTESIAN_POINT ( 'NONE',  ( -98.70698364546758796, -298.4791566786168460, -224.6489826538643229 ) ) ;
#39571=CARTESIAN_POINT ( 'NONE',  ( 15.46501485645788421, -274.4909083938114804, -219.8544147194975267 ) ) ;
#39572=CARTESIAN_POINT ( 'NONE',  ( 36.29268740888299050, -295.7352411305830628, -284.6081395539021628 ) ) ;
#39573=CARTESIAN_POINT ( 'NONE',  ( 38.78525149925633997, -287.5731310874433007, -258.7110261510833311 ) ) ;
#39574=CARTESIAN_POINT ( 'NONE',  ( -5.820619020157095314, -274.7817193097764630, -339.2576123025530705 ) ) ;
#39575=CARTESIAN_POINT ( 'NONE',  ( -105.1569721839799172, -289.9139449501035415, -306.8315015899572700 ) ) ;
#39576=CARTESIAN_POINT ( 'NONE',  ( 31.19903599478780620, -286.2660291231490532, -244.4191415195332979 ) ) ;
#39577=CARTESIAN_POINT ( 'NONE',  ( -95.02391647623375093, -289.2139908503600623, -222.4062975314594723 ) ) ;
#39580=CARTESIAN_POINT ( 'NONE',  ( 19.55746676059235867, -287.7072381380466481, -316.1920382139415437 ) ) ;
#39582=CARTESIAN_POINT ( 'NONE',  ( -112.7693390258945527, -285.6757783252675722, -255.8192634680230810 ) ) ;
#39583=CARTESIAN_POINT ( 'NONE',  ( 39.20733441517335649, -292.5387666794915731, -264.6108551255226189 ) ) ;
#39584=CARTESIAN_POINT ( 'NONE',  ( -19.95873125215370791, -281.8719504599476977, -196.1161337112993692 ) ) ;
#39585=CARTESIAN_POINT ( 'NONE',  ( -31.13060539442625796, -281.4441023927697074, -194.0544495326429058 ) ) ;
#39586=CARTESIAN_POINT ( 'NONE',  ( -53.69173315707597993, -283.1010384103417437, -341.5586623051245851 ) ) ;
#39587=CARTESIAN_POINT ( 'NONE',  ( 17.06581591602746428, -278.2765412748610743, -321.9830401343415360 ) ) ;
#39588=CARTESIAN_POINT ( 'NONE',  ( -106.5133198205408434, -296.9865379864292549, -236.5338061011563866 ) ) ;
#39589=CARTESIAN_POINT ( 'NONE',  ( -93.30008874856969214, -274.5406000743387835, -222.6981953964760237 ) ) ;
#39590=CARTESIAN_POINT ( 'NONE',  ( 28.95877907738960388, -291.1161866959914732, -236.0669018985278456 ) ) ;
#39591=UNCERTAINTY_MEASURE_WITH_UNIT (LENGTH_MEASURE( 1.000000000000000082E-05 ), #78729, 'distance_accuracy_value', 'NONE');
#39592=CARTESIAN_POINT ( 'NONE',  ( -84.26217448119713538, -296.3096047027069631, -213.9681678806313130 ) ) ;
#39595=CARTESIAN_POINT ( 'NONE',  ( -110.3458981331085482, -286.6605318393076232, -255.8111601022635568 ) ) ;
#39596=CARTESIAN_POINT ( 'NONE',  ( -24.94417792124987798, -295.9773838221981350, -346.0971585270480091 ) ) ;
#39597=CARTESIAN_POINT ( 'NONE',  ( -110.4114593512874194, -285.2321374479657834, -268.1924882522145026 ) ) ;
#39598=CARTESIAN_POINT ( 'NONE',  ( -4.107595489404640254, -275.6833631239210831, -339.5732192568361825 ) ) ;
#39599=CARTESIAN_POINT ( 'NONE',  ( -27.86988528739975379, -292.8206873134328134, -193.9950161240570594 ) ) ;
#39600=CARTESIAN_POINT ( 'NONE',  ( -7.802488213262869898, -284.5745774425386116, -200.5361680304797289 ) ) ;
#39602=CARTESIAN_POINT ( 'NONE',  ( -0.8176332796311546192, -292.8569861591918198, -202.5987624123526984 ) ) ;
#39603=CARTESIAN_POINT ( 'NONE',  ( -48.05989454545237294, -289.5254125194103949, -342.6423960824848791 ) ) ;
#39605=CARTESIAN_POINT ( 'NONE',  ( -109.5186219979625974, -268.8715237626327053, -295.3229297537549201 ) ) ;
#39606=CARTESIAN_POINT ( 'NONE',  ( -99.21482380618097352, -285.4737047574824942, -315.1083697265177079 ) ) ;
#39607=CARTESIAN_POINT ( 'NONE',  ( -19.05039376806006857, -277.7666405000204577, -190.3683826091709363 ) ) ;
#39608=ORIENTED_EDGE ( 'NONE', *, *, #37667, .T. ) ;
#39609=CARTESIAN_POINT ( 'NONE',  ( 33.94753095691120137, -280.6976765370531552, -287.5045854713155791 ) ) ;
#39610=CARTESIAN_POINT ( 'NONE',  ( -108.4914965712454915, -278.5924476445994173, -240.9765853583650141 ) ) ;
#39611=CARTESIAN_POINT ( 'NONE',  ( -6.024868469727883813, -282.4648206990967765, -202.3818130691016961 ) ) ;
#39612=CARTESIAN_POINT ( 'NONE',  ( 140.6027560640470142, 178.2755120123287611, -239.6641268871332500 ) ) ;
#39613=CARTESIAN_POINT ( 'NONE',  ( -61.06609947409423711, -281.9288151696048317, -343.0508027466426597 ) ) ;
#39614=CARTESIAN_POINT ( 'NONE',  ( 36.19206204641257330, -285.4029588444121259, -257.2380762053180661 ) ) ;
#39615=CARTESIAN_POINT ( 'NONE',  ( -75.29349592602395091, -299.3140378956080667, -204.4703696497196859 ) ) ;
#39616=CARTESIAN_POINT ( 'NONE',  ( -31.59126198278418940, -295.4700904781654458, -343.2461613136113669 ) ) ;
#39619=CARTESIAN_POINT ( 'NONE',  ( 17.11479098862842108, -291.5338982140329449, -220.9333012391132343 ) ) ;
#39620=CARTESIAN_POINT ( 'NONE',  ( -2.763504090707678884, -277.2585595331883610, -339.0610095549510561 ) ) ;
#39621=CARTESIAN_POINT ( 'NONE',  ( -51.56145966796525215, -273.8653203209354956, -198.7076633503091330 ) ) ;
#39622=CARTESIAN_POINT ( 'NONE',  ( 34.90511988341609850, -274.8002694296607729, -296.2447807844613976 ) ) ;
#39624=CARTESIAN_POINT ( 'NONE',  ( 27.62765049496321268, -273.0507116727614516, -232.7887045907048389 ) ) ;
#39625=CARTESIAN_POINT ( 'NONE',  ( -47.53486938215063873, -296.6045794102851119, -346.0889569348577766 ) ) ;
#39630=CARTESIAN_POINT ( 'NONE',  ( -82.97644637447366733, -284.7729323286050658, -327.7995511489230580 ) ) ;
#39631=CARTESIAN_POINT ( 'NONE',  ( -2.084156676595279478, -284.3519597862401724, -337.6729270923661375 ) ) ;
#39632=CARTESIAN_POINT ( 'NONE',  ( -82.86467103295676395, -283.0421262334570542, -327.6235596081834842 ) ) ;
#39633=CARTESIAN_POINT ( 'NONE',  ( 12.27060056339095517, -274.7480859062198988, -325.0661477351733879 ) ) ;
#39634=CARTESIAN_POINT ( 'NONE',  ( -53.94323939252092970, -285.1278082313111781, -342.7691370784489777 ) ) ;
#39635=CARTESIAN_POINT ( 'NONE',  ( -68.34658320717315405, -275.9468758556681109, -337.2286067586991294 ) ) ;
#39637=CARTESIAN_POINT ( 'NONE',  ( 34.19793077050955787, -276.8428787879513493, -286.4278464394835737 ) ) ;
#39640=CARTESIAN_POINT ( 'NONE',  ( -111.1849022949874524, -279.6219005887551248, -249.1163465217204021 ) ) ;
#39643=CARTESIAN_POINT ( 'NONE',  ( -77.88185896896445115, -287.3740828116817738, -206.3548604724969948 ) ) ;
#39644=CARTESIAN_POINT ( 'NONE',  ( -61.07519455262079333, -294.5653072566602191, -339.6197483953746428 ) ) ;
#39645=CARTESIAN_POINT ( 'NONE',  ( -80.49028880831879462, -288.9685695071562463, -334.0769388608529766 ) ) ;
#39646=CARTESIAN_POINT ( 'NONE',  ( 33.27376178377338789, -286.0837990396106534, -292.6997589782764635 ) ) ;
#39647=CARTESIAN_POINT ( 'NONE',  ( -19.65681778267361324, -284.8587748896123344, -198.9284934201445196 ) ) ;
#39648=CARTESIAN_POINT ( 'NONE',  ( -52.55648522724863625, -290.0945818635508431, -197.8758809785319386 ) ) ;
#39649=CARTESIAN_POINT ( 'NONE',  ( -85.10863555245676082, -284.9342144054907067, -326.0876860077471520 ) ) ;
#39650=CARTESIAN_POINT ( 'NONE',  ( -9.966185078670209307, -274.6945206846938277, -340.1864846127739384 ) ) ;
#39651=CARTESIAN_POINT ( 'NONE',  ( -57.10328329638918632, -287.7026815511279096, -344.0085911247178387 ) ) ;
#39652=CARTESIAN_POINT ( 'NONE',  ( -8.145820723512962047, -288.4345302531881430, -201.2219278970269158 ) ) ;
#39653=CARTESIAN_POINT ( 'NONE',  ( 34.93560693069736089, -285.2848066327330798, -249.5358395156733593 ) ) ;
#39654=CARTESIAN_POINT ( 'NONE',  ( -13.44128764559060585, -283.6754403573763170, -339.6404627502159315 ) ) ;
#39655=CARTESIAN_POINT ( 'NONE',  ( -7.620811099606910943, -290.6636682921705415, -339.4162931606959432 ) ) ;
#39659=CARTESIAN_POINT ( 'NONE',  ( -88.64879474235468138, -299.2595524808058371, -214.8204408018097524 ) ) ;
#39661=CARTESIAN_POINT ( 'NONE',  ( -30.04307726684865543, -278.1442228730077773, -195.6653560981789894 ) ) ;
#39662=CARTESIAN_POINT ( 'NONE',  ( 8.762224741406479112, -291.8630777705416222, -208.8244934466491998 ) ) ;
#39663=CARTESIAN_POINT ( 'NONE',  ( -110.8983861085746128, -294.8660274973246374, -276.9510221037945144 ) ) ;
#39664=CARTESIAN_POINT ( 'NONE',  ( 34.12580315037016021, -280.4622120882492595, -287.5505193294093829 ) ) ;
#39665=CARTESIAN_POINT ( 'NONE',  ( -32.57486717372825780, -272.1925185161367153, -196.0611216984173382 ) ) ;
#39666=CARTESIAN_POINT ( 'NONE',  ( -9.025499807376524686, -295.9890977240772827, -338.1939611895390385 ) ) ;
#39667=CARTESIAN_POINT ( 'NONE',  ( 22.62177241418591933, -301.3029683736232300, -195.3356572496892625 ) ) ;
#39668=CARTESIAN_POINT ( 'NONE',  ( -87.63479199453202284, -271.9410463940280351, -212.7650420924811669 ) ) ;
#39669=CARTESIAN_POINT ( 'NONE',  ( 36.11120101886904621, -292.0388766214174439, -289.8199290694760180 ) ) ;
#39672=CARTESIAN_POINT ( 'NONE',  ( 35.69517182657597232, -294.2883065242595535, -265.2949977014166052 ) ) ;
#39675=CARTESIAN_POINT ( 'NONE',  ( -19.33637210163773901, -280.8418754809615621, -343.5873989137619446 ) ) ;
#39676=CARTESIAN_POINT ( 'NONE',  ( -34.30119463534659019, -295.0128625237863957, -343.2977708146487998 ) ) ;
#39677=CARTESIAN_POINT ( 'NONE',  ( 17.82627695980227500, -282.2893252683851415, -324.1541018679840249 ) ) ;
#39678=CARTESIAN_POINT ( 'NONE',  ( -113.5790427396694042, -284.0808196680319497, -281.3966533056985213 ) ) ;
#39679=CARTESIAN_POINT ( 'NONE',  ( -110.1396696716633130, -288.3289069964955615, -287.6955940677410695 ) ) ;
#39680=CARTESIAN_POINT ( 'NONE',  ( -27.48105051923313980, -281.4090623402646543, -346.0808686061739650 ) ) ;
#39681=CARTESIAN_POINT ( 'NONE',  ( -26.20308914757249497, -287.8338521637489862, -346.2388080799579484 ) ) ;
#39683=CARTESIAN_POINT ( 'NONE',  ( -50.59509220362742354, -296.8243748854167734, -342.9613109005114779 ) ) ;
#39684=CARTESIAN_POINT ( 'NONE',  ( 3.204342167205097791, -277.9444558263751333, -335.1893331159667468 ) ) ;
#39685=CARTESIAN_POINT ( 'NONE',  ( -107.2461319274750338, -278.4982249338487463, -249.2552443545260417 ) ) ;
#39686=CARTESIAN_POINT ( 'NONE',  ( -7.192158773138485728, -292.6035089675882546, -199.4948017430098730 ) ) ;
#39687=CARTESIAN_POINT ( 'NONE',  ( -88.88572816199265958, -283.4151340673147388, -215.0402960077908574 ) ) ;
#39688=CARTESIAN_POINT ( 'NONE',  ( -70.65889170467927727, -279.4917056388626975, -337.5546102152597427 ) ) ;
#39689=CARTESIAN_POINT ( 'NONE',  ( 35.43936246825725789, -292.7238329486046950, -278.9499967125762510 ) ) ;
#39691=CARTESIAN_POINT ( 'NONE',  ( -98.28124022598166221, -295.1468274312157973, -226.6418647505824140 ) ) ;
#39695=CARTESIAN_POINT ( 'NONE',  ( 35.76953186481645730, -293.0651450879711319, -270.7665164003734617 ) ) ;
#39697=CARTESIAN_POINT ( 'NONE',  ( -109.1418805571601069, -294.0523547857346784, -270.3284710469131937 ) ) ;
#39698=CARTESIAN_POINT ( 'NONE',  ( 19.18545054807930228, -297.8023799065100548, -193.6051735408791785 ) ) ;
#39700=CARTESIAN_POINT ( 'NONE',  ( 1.258312855294479782, -287.8715244392993213, -204.2903176100155065 ) ) ;
#39701=CARTESIAN_POINT ( 'NONE',  ( -88.66257608494407805, -289.6306402131138498, -322.2761225141631485 ) ) ;
#39703=CARTESIAN_POINT ( 'NONE',  ( -110.1743798349186676, -279.9255328864710464, -281.5909229495017030 ) ) ;
#39704=CARTESIAN_POINT ( 'NONE',  ( -72.16127415136023160, -299.3451779327166378, -205.0353799725195927 ) ) ;
#39705=CARTESIAN_POINT ( 'NONE',  ( -70.64661801114796447, -276.2965246263129870, -335.7668742335099523 ) ) ;
#39707=CARTESIAN_POINT ( 'NONE',  ( -109.1658334348097270, -272.7386872876663801, -242.4601928849913008 ) ) ;
#39708=CARTESIAN_POINT ( 'NONE',  ( -93.48193564286293622, -291.7880724401666725, -319.3215310150362143 ) ) ;
#39709=CARTESIAN_POINT ( 'NONE',  ( 34.68962801281556096, -294.8338191310930370, -245.3433624781305582 ) ) ;
#39710=CARTESIAN_POINT ( 'NONE',  ( -113.1465174729249270, -274.3934560397275391, -270.3845621914958883 ) ) ;
#39711=CARTESIAN_POINT ( 'NONE',  ( -107.8523963470944409, -291.4580801992955230, -251.0703329511936772 ) ) ;
#39714=CARTESIAN_POINT ( 'NONE',  ( 10.35979044841188035, -290.8416062541252813, -211.4304278360350793 ) ) ;
#39715=CARTESIAN_POINT ( 'NONE',  ( -51.80080555010563614, -298.2054241824904466, -194.6980728815351540 ) ) ;
#39716=CARTESIAN_POINT ( 'NONE',  ( -41.86541348196897872, -297.6602956599268168, -197.4802322559225445 ) ) ;
#39719=CARTESIAN_POINT ( 'NONE',  ( -90.31864062599562715, -292.8394148066545313, -215.3682653294903275 ) ) ;
#39720=CARTESIAN_POINT ( 'NONE',  ( 36.57525178469696669, -289.6233781216987495, -234.7283546768995564 ) ) ;
#39721=CARTESIAN_POINT ( 'NONE',  ( -110.7318193497294345, -286.7405253257752520, -255.7351537302855888 ) ) ;
#39722=CARTESIAN_POINT ( 'NONE',  ( 23.79292097534147032, -272.9641282565760889, -227.1812320932447165 ) ) ;
#39723=CARTESIAN_POINT ( 'NONE',  ( -67.66607105041461523, -275.5713059889473584, -202.3637226577957051 ) ) ;
#39724=CARTESIAN_POINT ( 'NONE',  ( 9.778903110907036123, -290.7860816474361627, -212.6664447397970150 ) ) ;
#39725=CARTESIAN_POINT ( 'NONE',  ( -111.7870033245331172, -280.5923878887890623, -256.2131863788128499 ) ) ;
#39727=CARTESIAN_POINT ( 'NONE',  ( -51.04512795253646829, -282.5803749545330561, -342.2188167373320766 ) ) ;
#39728=CARTESIAN_POINT ( 'NONE',  ( -109.4414312862656686, -279.2986155744231382, -296.6529795015550235 ) ) ;
#39729=CARTESIAN_POINT ( 'NONE',  ( -17.08216137139889312, -279.1030095750335249, -196.4858189516522771 ) ) ;
#39730=CARTESIAN_POINT ( 'NONE',  ( 137.1993315682407513, 179.5396152623583816, -238.8328485414318436 ) ) ;
#39731=CARTESIAN_POINT ( 'NONE',  ( 35.84194613142251740, -276.7855449304253170, -293.5338203081345227 ) ) ;
#39733=CARTESIAN_POINT ( 'NONE',  ( -32.74389777622274522, -275.6291922407170887, -194.1800611126437843 ) ) ;
#39734=CARTESIAN_POINT ( 'NONE',  ( -54.49178911615187815, -300.3376638359845856, -195.3683826091709363 ) ) ;
#39736=VERTEX_POINT ( 'NONE', #27857 ) ;
#39738=CARTESIAN_POINT ( 'NONE',  ( -31.83446811926402731, -290.0608417822717229, -343.5139151645066136 ) ) ;
#39739=CARTESIAN_POINT ( 'NONE',  ( 22.50343835863060704, -289.9466763791970152, -317.2065722804399002 ) ) ;
#39740=CARTESIAN_POINT ( 'NONE',  ( -86.80444592184629471, -289.1103571408332300, -324.2566429272066557 ) ) ;
#39741=CARTESIAN_POINT ( 'NONE',  ( -15.42497997227498630, -285.8359702797824866, -196.5549427593896894 ) ) ;
#39743=CARTESIAN_POINT ( 'NONE',  ( -18.55140352823800853, -281.2060668890777606, -341.7819079804012290 ) ) ;
#39744=CARTESIAN_POINT ( 'NONE',  ( 34.27982309166126385, -289.6684566812014623, -290.0770342393511214 ) ) ;
#39745=CARTESIAN_POINT ( 'NONE',  ( -65.59928976714695636, -281.9083649889072944, -338.4352352226174503 ) ) ;
#39746=CARTESIAN_POINT ( 'NONE',  ( -87.88183246933533610, -280.6432015741103783, -216.9340625338751067 ) ) ;
#39747=CARTESIAN_POINT ( 'NONE',  ( 37.27853583509865842, -288.7200889668467312, -288.4344708695062423 ) ) ;
#39748=CARTESIAN_POINT ( 'NONE',  ( -39.15300923662992005, -277.5678422768293672, -343.4002006790905170 ) ) ;
#39749=CARTESIAN_POINT ( 'NONE',  ( -95.35013347247358695, -290.0263799320351836, -220.3107788947947370 ) ) ;
#39750=CARTESIAN_POINT ( 'NONE',  ( -63.15682724680156213, -286.5271062904726591, -197.9888993338646799 ) ) ;
#39751=CARTESIAN_POINT ( 'NONE',  ( -40.81997165677712758, -286.5019795035723291, -193.4491690200500784 ) ) ;
#39752=CARTESIAN_POINT ( 'NONE',  ( -37.53839109535314833, -283.2213979392259375, -343.3732823468525908 ) ) ;
#39755=CARTESIAN_POINT ( 'NONE',  ( -110.7197263458815257, -292.1720032796042119, -289.2801411478302498 ) ) ;
#39757=CARTESIAN_POINT ( 'NONE',  ( -0.9555650506191690763, -293.2643335911649274, -337.6763333024496774 ) ) ;
#39758=CARTESIAN_POINT ( 'NONE',  ( -32.66406834142569693, -273.1712625433654011, -197.2627920962744952 ) ) ;
#39760=CARTESIAN_POINT ( 'NONE',  ( -65.57380561601503643, -294.7603512162481820, -341.9033653222387557 ) ) ;
#39761=CARTESIAN_POINT ( 'NONE',  ( -93.06822552151373884, -289.7127123954507510, -222.1401461826363288 ) ) ;
#39762=CARTESIAN_POINT ( 'NONE',  ( -96.42663509871108829, -294.1742092870052829, -314.9571589436030763 ) ) ;
#39764=CARTESIAN_POINT ( 'NONE',  ( -101.4780791103513593, -292.2438030974962544, -234.5683815685820548 ) ) ;
#39767=CARTESIAN_POINT ( 'NONE',  ( 36.26989864591389079, -291.7468634837658783, -285.5716720862241687 ) ) ;
#39768=CARTESIAN_POINT ( 'NONE',  ( -34.05362665422288160, -297.0110893642420820, -345.3392244205235784 ) ) ;
#39769=CARTESIAN_POINT ( 'NONE',  ( 33.93655589983130483, -288.2715593302011712, -253.4897439839930371 ) ) ;
#39770=CONICAL_SURFACE ( 'NONE', #3509, 2.395975569037533948, 0.09862129276975308001 ) ;
#39771=CARTESIAN_POINT ( 'NONE',  ( 0.2488915315052253607, -278.5344535952655178, -335.7299933199262227 ) ) ;
#39772=CARTESIAN_POINT ( 'NONE',  ( -6.747456131714818284, -275.4543248688745507, -340.6035053402041513 ) ) ;
#39773=CARTESIAN_POINT ( 'NONE',  ( -29.07093834134551713, -297.3504034485424086, -193.5236867680119133 ) ) ;
#39774=CARTESIAN_POINT ( 'NONE',  ( -10.91284753882835190, -274.9426332593550342, -339.4949719501360619 ) ) ;
#39775=CARTESIAN_POINT ( 'NONE',  ( -95.04150366694798890, -277.2849096088735337, -223.3287156075291762 ) ) ;
#39776=CARTESIAN_POINT ( 'NONE',  ( -41.36281958430816275, -275.5018334940079967, -346.4680198426538027 ) ) ;
#39780=CARTESIAN_POINT ( 'NONE',  ( -63.35073241327500426, -274.3555528266676333, -202.0290649443586801 ) ) ;
#39782=CARTESIAN_POINT ( 'NONE',  ( -10.18022559315754982, -286.7194527106200326, -340.6509544034244072 ) ) ;
#39783=CARTESIAN_POINT ( 'NONE',  ( -29.98775596008918853, -273.9811398031532690, -197.7324768712551304 ) ) ;
#39785=CARTESIAN_POINT ( 'NONE',  ( 39.34744552469121004, -287.6385955382169755, -277.2730597537149038 ) ) ;
#39786=CARTESIAN_POINT ( 'NONE',  ( -35.54682324546423189, -300.0544014925458782, -195.0053073947756559 ) ) ;
#39787=CARTESIAN_POINT ( 'NONE',  ( -89.80486420785283030, -293.7939382221726419, -323.7972950000556125 ) ) ;
#39788=CARTESIAN_POINT ( 'NONE',  ( 33.41323309201952441, -281.1330312446541484, -300.4619046728660123 ) ) ;
#39790=CARTESIAN_POINT ( 'NONE',  ( -26.48868791700703440, -278.1899538328263475, -196.0989576444739271 ) ) ;
#39793=CARTESIAN_POINT ( 'NONE',  ( -108.1127691114707545, -289.0891583803602884, -290.0058528152225676 ) ) ;
#39796=CARTESIAN_POINT ( 'NONE',  ( -47.23371169119993596, -289.9262888776588625, -196.0163215659109710 ) ) ;
#39797=CARTESIAN_POINT ( 'NONE',  ( -43.55974445737484047, -275.4924468666928874, -196.8793887419329849 ) ) ;
#39798=CARTESIAN_POINT ( 'NONE',  ( -4.401282570986539078, -284.0517898906515484, -339.3213841356649141 ) ) ;
#39799=CARTESIAN_POINT ( 'NONE',  ( -107.8145378871846987, -270.9854956299136575, -242.9611489228998380 ) ) ;
#39800=CARTESIAN_POINT ( 'NONE',  ( -24.06549518659920039, -282.8778344105186306, -342.1437229948592744 ) ) ;
#39801=CARTESIAN_POINT ( 'NONE',  ( 15.86032821095262690, -276.2491782610504174, -219.4452743736653417 ) ) ;
#39802=CARTESIAN_POINT ( 'NONE',  ( 34.86821958725052895, -276.5138298591160151, -282.4288300823610030 ) ) ;
#39803=CARTESIAN_POINT ( 'NONE',  ( -46.97361172118782946, -285.1746618732933598, -344.7400593985273645 ) ) ;
#39804=CARTESIAN_POINT ( 'NONE',  ( -40.51621138919293941, -297.0700364246780509, -197.1820682965733624 ) ) ;
#39807=CARTESIAN_POINT ( 'NONE',  ( 38.32563184522916799, -293.2070849189560704, -256.0973570282072842 ) ) ;
#39808=CARTESIAN_POINT ( 'NONE',  ( -96.40272711318992549, -285.9032532665411850, -316.0289007689420941 ) ) ;
#39810=CARTESIAN_POINT ( 'NONE',  ( -88.52914483777347243, -275.1952119285919025, -334.4957818155094174 ) ) ;
#39811=CARTESIAN_POINT ( 'NONE',  ( -113.8820721935425695, -277.8413357026964263, -263.0191635710657465 ) ) ;
#39812=CARTESIAN_POINT ( 'NONE',  ( -113.3881522850110173, -289.0131285028289767, -265.5260866407580806 ) ) ;
#39813=CARTESIAN_POINT ( 'NONE',  ( -33.44034290159669354, -284.5223116261956875, -343.9638035118141488 ) ) ;
#39814=CARTESIAN_POINT ( 'NONE',  ( -35.06430666747245084, -278.7833057854938374, -344.3394086807946906 ) ) ;
#39815=CARTESIAN_POINT ( 'NONE',  ( -46.45337606932299224, -287.3639393147903434, -194.4955549543988980 ) ) ;
#39816=CARTESIAN_POINT ( 'NONE',  ( -27.31555767499168041, -282.1795958621367504, -195.9817001519840858 ) ) ;
#39817=CARTESIAN_POINT ( 'NONE',  ( 31.24933441125983435, -275.2681994449073954, -235.3715483180508272 ) ) ;
#39818=CARTESIAN_POINT ( 'NONE',  ( -28.60314493002260150, -276.7776896760775003, -346.9172268872580958 ) ) ;
#39819=CONICAL_SURFACE ( 'NONE', #11124, 2.395975569037533948, 0.09862129276975308001 ) ;
#39820=CARTESIAN_POINT ( 'NONE',  ( -89.49359142643116627, -297.7136211299420552, -323.5512755501623587 ) ) ;
#39823=CARTESIAN_POINT ( 'NONE',  ( -51.54544036838969845, -296.0120801104989141, -195.8861563920898732 ) ) ;
#39824=CARTESIAN_POINT ( 'NONE',  ( -100.6392797531233327, -277.5587018973620843, -306.9511625713876128 ) ) ;
#39825=CARTESIAN_POINT ( 'NONE',  ( -31.30673008393911871, -275.3318181946322056, -193.9830712550185012 ) ) ;
#39826=CARTESIAN_POINT ( 'NONE',  ( 36.13283947421767550, -289.4282842924586134, -279.2754908239335805 ) ) ;
#39827=CARTESIAN_POINT ( 'NONE',  ( -41.88475481592588778, -296.6284003057389782, -346.5843498001004832 ) ) ;
#39828=CARTESIAN_POINT ( 'NONE',  ( -113.9135278707518637, -297.8023800467317983, -266.7692820837592080 ) ) ;
#39829=CARTESIAN_POINT ( 'NONE',  ( -112.1375019110005269, -292.5051888326643734, -274.0234576335558359 ) ) ;
#39830=CARTESIAN_POINT ( 'NONE',  ( -54.89881208862858841, -277.8258897682926545, -197.5630188277108630 ) ) ;
#39832=CARTESIAN_POINT ( 'NONE',  ( 5.736976495290038613, -282.5612118126936707, -209.6524545500743670 ) ) ;
#39833=CARTESIAN_POINT ( 'NONE',  ( -105.0177499493420612, -295.0435134676999951, -239.2328409918157490 ) ) ;
#39834=CARTESIAN_POINT ( 'NONE',  ( -68.65398484356734343, -285.3196887404208724, -339.3669378444746485 ) ) ;
#39835=CARTESIAN_POINT ( 'NONE',  ( 33.33090819253290960, -286.2161143851173506, -250.8775734543809506 ) ) ;
#39836=CARTESIAN_POINT ( 'NONE',  ( -54.34854212782089178, -170.4010203859631645, -363.8413129607317273 ) ) ;
#39838=CARTESIAN_POINT ( 'NONE',  ( 34.01757299924511813, -287.0145897466731526, -254.8710687375991313 ) ) ;
#39840=CARTESIAN_POINT ( 'NONE',  ( -30.22981603279387031, -284.0438337334412608, -346.7215371418542418 ) ) ;
#39842=CARTESIAN_POINT ( 'NONE',  ( -81.08706607163028934, -273.7728029653857220, -211.8303224405265155 ) ) ;
#39843=CARTESIAN_POINT ( 'NONE',  ( -2.390312730128070662, -285.2990705822073778, -202.1818655209577003 ) ) ;
#39845=CARTESIAN_POINT ( 'NONE',  ( 10.66648957686888366, -281.6380748477394036, -210.3927946783440177 ) ) ;
#39847=CARTESIAN_POINT ( 'NONE',  ( -59.12292222997164259, -281.2953699237994556, -197.2291406064128694 ) ) ;
#39848=CARTESIAN_POINT ( 'NONE',  ( 38.85094398147693084, -282.0227129027796309, -281.3349630293132577 ) ) ;
#39849=CARTESIAN_POINT ( 'NONE',  ( 30.89617123739170168, -285.2666405000203440, -285.9686137636504668 ) ) ;
#39850=CARTESIAN_POINT ( 'NONE',  ( -47.70296038983430265, -155.1840385668599538, -365.3184360848422898 ) ) ;
#39852=CARTESIAN_POINT ( 'NONE',  ( -9.277769870770052663, -278.6846286850316119, -339.7468093962818898 ) ) ;
#39853=CARTESIAN_POINT ( 'NONE',  ( 198.8369974573453192, 289.4883165844757968, -97.36247972072811763 ) ) ;
#39855=CARTESIAN_POINT ( 'NONE',  ( 37.06645056988301690, -279.6568738698627499, -276.9202094849629816 ) ) ;
#39856=CARTESIAN_POINT ( 'NONE',  ( -4.914356814633031867, -296.3911815409174437, -339.0954218122809607 ) ) ;
#39857=CARTESIAN_POINT ( 'NONE',  ( -55.83709986365592215, -294.6450891098947977, -341.1370720201487643 ) ) ;
#39858=CARTESIAN_POINT ( 'NONE',  ( -111.1713454743743341, -290.3315761753734705, -248.7113980921081122 ) ) ;
#39860=CARTESIAN_POINT ( 'NONE',  ( -112.0330643881362107, -294.9237475370731545, -286.4796290860215890 ) ) ;
#39861=CARTESIAN_POINT ( 'NONE',  ( 32.14587634846064645, -286.2794187540621920, -295.2190569507674240 ) ) ;
#39862=CARTESIAN_POINT ( 'NONE',  ( 20.67368585677700565, -296.0560761843204318, -316.6964045232886633 ) ) ;
#39863=CARTESIAN_POINT ( 'NONE',  ( -107.4513170884046076, -285.5771229778363249, -292.4039192537188114 ) ) ;
#39865=CARTESIAN_POINT ( 'NONE',  ( 22.91589289952115038, -293.8551077152234825, -222.7812833551403457 ) ) ;
#39866=CARTESIAN_POINT ( 'NONE',  ( -104.6566933204832281, -285.4269383999828733, -241.8289387030356750 ) ) ;
#39867=CARTESIAN_POINT ( 'NONE',  ( -81.65457398396021915, -294.4352005469737605, -332.9109350206140334 ) ) ;
#39869=CARTESIAN_POINT ( 'NONE',  ( -113.8470875312444406, -291.4514566630433023, -262.6633235361706511 ) ) ;
#39870=CARTESIAN_POINT ( 'NONE',  ( -107.2071811897092601, -291.4584643097590515, -238.0108554379469012 ) ) ;
#39871=CARTESIAN_POINT ( 'NONE',  ( -42.66179500164579252, -289.2876755957583441, -343.2176048613244461 ) ) ;
#39874=CARTESIAN_POINT ( 'NONE',  ( 7.062238062185569376, -300.4628266708469368, -194.5824113571880503 ) ) ;
#39875=CARTESIAN_POINT ( 'NONE',  ( -49.64028476192080319, -272.6937164334059958, -194.6983753253464897 ) ) ;
#39876=CARTESIAN_POINT ( 'NONE',  ( -51.86232481402274885, -278.9206433638852332, -198.5278881975040122 ) ) ;
#39879=CARTESIAN_POINT ( 'NONE',  ( 11.75125115413071164, -274.2202303522391844, -211.0516182497405850 ) ) ;
#39880=CARTESIAN_POINT ( 'NONE',  ( -97.43702802450373213, -295.6220396974227356, -227.7083417737426316 ) ) ;
#39881=CARTESIAN_POINT ( 'NONE',  ( -95.40457104334377902, -279.7699491780040830, -316.6368852998749617 ) ) ;
#39882=CARTESIAN_POINT ( 'NONE',  ( 12.39131684248492959, -272.8926628506566203, -215.1784298547269429 ) ) ;
#39883=CARTESIAN_POINT ( 'NONE',  ( -95.61362895822911412, -298.3818479192134987, -225.7142651774272508 ) ) ;
#39884=CARTESIAN_POINT ( 'NONE',  ( -107.0048185663945475, -297.9354740795042176, -247.3686203846012575 ) ) ;
#39886=CARTESIAN_POINT ( 'NONE',  ( -110.8557563086801849, -298.4082980940353309, -250.1129179588720888 ) ) ;
#39887=CARTESIAN_POINT ( 'NONE',  ( -96.50567071643585848, -271.2101287116694266, -223.6917341026262704 ) ) ;
#39888=CARTESIAN_POINT ( 'NONE',  ( 33.21726461501619099, -294.4562650530234578, -289.5222139637552345 ) ) ;
#39889=CARTESIAN_POINT ( 'NONE',  ( 22.29277605024654463, -291.5282874515282856, -227.2223528185431576 ) ) ;
#39890=FACE_OUTER_BOUND ( 'NONE', #45668, .T. ) ;
#39891=CARTESIAN_POINT ( 'NONE',  ( 22.70638377164603483, -275.3994269881756622, -222.2387259433414499 ) ) ;
#39892=CARTESIAN_POINT ( 'NONE',  ( -60.52663324946901469, -298.0764108567388462, -201.0649693514104683 ) ) ;
#39893=CARTESIAN_POINT ( 'NONE',  ( 34.59780140026816042, -283.2441020441747241, -247.9308945565724684 ) ) ;
#39894=CARTESIAN_POINT ( 'NONE',  ( -76.51984852833768969, -282.2491880421223414, -336.1368618603453911 ) ) ;
#39895=CARTESIAN_POINT ( 'NONE',  ( -75.29312218112123389, -276.8929762310203841, -337.2416259860366949 ) ) ;
#39897=CARTESIAN_POINT ( 'NONE',  ( -64.12398131338626683, -282.6078747705284968, -338.4442373411538370 ) ) ;
#39898=CARTESIAN_POINT ( 'NONE',  ( 26.72865974338654382, -280.0792582641491322, -309.7664139892644926 ) ) ;
#39900=CARTESIAN_POINT ( 'NONE',  ( 17.86534855371302655, -274.8163437526249595, -319.0376675416437706 ) ) ;
#39901=CARTESIAN_POINT ( 'NONE',  ( -10.66344824300929162, -278.7044963706738940, -340.5099735875199940 ) ) ;
#39904=CARTESIAN_POINT ( 'NONE',  ( -103.5244894767228203, -271.4489132294216347, -232.4891674483793338 ) ) ;
#39906=CARTESIAN_POINT ( 'NONE',  ( -102.0150896752214464, -280.0399051690092165, -308.7695419381665829 ) ) ;
#39908=CARTESIAN_POINT ( 'NONE',  ( -82.99336479221003060, -285.5910860038545707, -330.6367910575937117 ) ) ;
#39911=CARTESIAN_POINT ( 'NONE',  ( 8.286716363009247743, -286.4281190546503808, -329.9493301367932077 ) ) ;
#39913=CARTESIAN_POINT ( 'NONE',  ( -80.40005331173402681, -294.4453725542026064, -329.8010769738037311 ) ) ;
#39914=CARTESIAN_POINT ( 'NONE',  ( -72.97218697348505145, -287.6692207758283644, -335.4866420795630688 ) ) ;
#39916=CARTESIAN_POINT ( 'NONE',  ( -102.9521984419405385, -295.0353824857957079, -234.0256923327315803 ) ) ;
#39917=CARTESIAN_POINT ( 'NONE',  ( -60.28286420397969891, -284.2400137719881741, -197.5296040163914029 ) ) ;
#39918=CARTESIAN_POINT ( 'NONE',  ( 31.81288479365725763, -282.8105580342979692, -244.4447926933517579 ) ) ;
#39919=CARTESIAN_POINT ( 'NONE',  ( 10.83262658920518540, -280.6366957417903905, -329.1931955109091064 ) ) ;
#39920=CARTESIAN_POINT ( 'NONE',  ( -98.11067330276347320, -289.9903813939259862, -310.8330020887377145 ) ) ;
#39921=AXIS2_PLACEMENT_3D ( 'NONE', #45863, #44474, #80932 ) ;
#39923=CARTESIAN_POINT ( 'NONE',  ( -108.1904886280531599, -280.2388526553801853, -250.4190437213241864 ) ) ;
#39924=CARTESIAN_POINT ( 'NONE',  ( -32.96354380183094435, -280.9115548554800625, -197.3307580329334314 ) ) ;
#39925=CARTESIAN_POINT ( 'NONE',  ( 31.37552165241656255, -289.9356616415514054, -301.2860307649806941 ) ) ;
#39928=CARTESIAN_POINT ( 'NONE',  ( -34.10319493175585848, -274.0918282862901378, -193.4292514765836017 ) ) ;
#39929=CARTESIAN_POINT ( 'NONE',  ( -109.3450010223550350, -292.7863444923192446, -250.6793633558575038 ) ) ;
#39930=CARTESIAN_POINT ( 'NONE',  ( 120.8395553409046528, -299.5541904835127980, -195.3611179825600175 ) ) ;
#39931=CARTESIAN_POINT ( 'NONE',  ( -37.30987171927208124, -297.5519495502701375, -350.3611179825600175 ) ) ;
#39932=EDGE_LOOP ( 'NONE', ( #57835, #77377 ) ) ;
#39933=CARTESIAN_POINT ( 'NONE',  ( 36.42460406899568426, -273.3669764058590204, -255.9194839109920565 ) ) ;
#39935=CARTESIAN_POINT ( 'NONE',  ( -88.08801166768149926, -294.1478237462674770, -327.2759970417426416 ) ) ;
#39936=CARTESIAN_POINT ( 'NONE',  ( -64.59910141930529903, -273.0352558882165113, -202.5174885453004663 ) ) ;
#39937=CARTESIAN_POINT ( 'NONE',  ( -71.47688267531636086, -291.0316460661204587, -335.6861459932318326 ) ) ;
#39938=CIRCLE ( 'NONE', #92888, 0.5000000000000004441 ) ;
#39939=CARTESIAN_POINT ( 'NONE',  ( -40.25207304407012288, -284.8493794377538393, -344.3172113402604282 ) ) ;
#39940=CARTESIAN_POINT ( 'NONE',  ( -73.17359136916491025, -293.0119222085804154, -202.8579474814561650 ) ) ;
#39941=CARTESIAN_POINT ( 'NONE',  ( -73.21738478106122727, -292.9018417216164494, -202.7724006240360666 ) ) ;
#39942=CARTESIAN_POINT ( 'NONE',  ( -9.725509357622222240, -292.2564084769883266, -202.7325883287784620 ) ) ;
#39943=CARTESIAN_POINT ( 'NONE',  ( -47.00718327411643571, -287.9296857594567314, -195.9343640610834427 ) ) ;
#39944=CARTESIAN_POINT ( 'NONE',  ( 39.41153979145496322, -281.6417979951140751, -264.2015590417603903 ) ) ;
#39945=CARTESIAN_POINT ( 'NONE',  ( -112.1721864685637087, -294.7666823356152577, -259.7933638427709298 ) ) ;
#39946=CARTESIAN_POINT ( 'NONE',  ( -34.48109616090975038, -282.8504461847399511, -347.3079629436462596 ) ) ;
#39947=CARTESIAN_POINT ( 'NONE',  ( 31.68645494205470214, -277.1581030884285610, -241.8184552063757451 ) ) ;
#39948=CARTESIAN_POINT ( 'NONE',  ( -21.33282851196159058, -291.3376638359844719, -340.3538533559490702 ) ) ;
#39949=CARTESIAN_POINT ( 'NONE',  ( -48.33850316556904403, -275.3301231220715977, -345.3766458612280985 ) ) ;
#39951=CARTESIAN_POINT ( 'NONE',  ( 1.128384709536257580, -282.0314394668641853, -332.5333217831845332 ) ) ;
#39952=CARTESIAN_POINT ( 'NONE',  ( -111.7041864223648417, -279.9890994613726320, -251.9162434612984782 ) ) ;
#39953=CARTESIAN_POINT ( 'NONE',  ( 21.30149730118791851, -287.2803279334011677, -319.8969192676487978 ) ) ;
#39954=CARTESIAN_POINT ( 'NONE',  ( -22.55985524192942648, -294.0041234129637360, -197.8389070902159403 ) ) ;
#39955=CARTESIAN_POINT ( 'NONE',  ( 32.96744214091626901, -276.7731805041838129, -240.8469596105385619 ) ) ;
#39956=CARTESIAN_POINT ( 'NONE',  ( 37.11583154547785313, -277.0893658874636571, -288.0066386532004685 ) ) ;
#39957=CARTESIAN_POINT ( 'NONE',  ( -36.46830422599426669, -276.8742602266501081, -343.3683603301077483 ) ) ;
#39958=CARTESIAN_POINT ( 'NONE',  ( -83.08440284735091552, -299.4249573799679069, -211.0701488321134889 ) ) ;
#39959=CARTESIAN_POINT ( 'NONE',  ( -110.7218213990089595, -282.7408513039162585, -255.6850751936578376 ) ) ;
#39960=CARTESIAN_POINT ( 'NONE',  ( 22.19560467496934208, -292.5634420680644325, -221.5650768682015155 ) ) ;
#39961=CARTESIAN_POINT ( 'NONE',  ( -23.43769816913287229, -290.4775242474386232, -345.3354248793496595 ) ) ;
#39962=CARTESIAN_POINT ( 'NONE',  ( -4.683071405612477811, -291.4130872516424802, -204.7145191384604459 ) ) ;
#39964=CARTESIAN_POINT ( 'NONE',  ( -58.75602935051295361, -290.3551797664517267, -197.0124111400807010 ) ) ;
#39965=CARTESIAN_POINT ( 'NONE',  ( 6.692368853513653626, -292.3367851412401137, -212.1108969048224253 ) ) ;
#39967=CARTESIAN_POINT ( 'NONE',  ( -28.99709303471507482, -290.0285433223718314, -346.6499859984701857 ) ) ;
#39968=CARTESIAN_POINT ( 'NONE',  ( -107.7186955520845686, -279.4651185866747483, -250.5417127838931322 ) ) ;
#39970=CARTESIAN_POINT ( 'NONE',  ( -111.6724675631351005, -295.2346947412398777, -289.2935132128879445 ) ) ;
#39971=CARTESIAN_POINT ( 'NONE',  ( -18.21541169642240732, -286.9436573448576837, -195.8245628828794054 ) ) ;
#39973=CARTESIAN_POINT ( 'NONE',  ( 2.726382592704248431, -286.9075092234311910, -204.6321818997711830 ) ) ;
#39974=CARTESIAN_POINT ( 'NONE',  ( -96.59446676261966047, -285.4822789304688513, -227.6642990782339950 ) ) ;
#39975=CARTESIAN_POINT ( 'NONE',  ( -13.18397878099063014, -91.46032863585759287, -359.9971981747313521 ) ) ;
#39976=CARTESIAN_POINT ( 'NONE',  ( 201.5604602716146871, 295.4035874922714697, -68.51738880406409749 ) ) ;
#39977=CARTESIAN_POINT ( 'NONE',  ( 166.7545789058513037, 230.2666759795009739, -189.9084627180601501 ) ) ;
#39978=CARTESIAN_POINT ( 'NONE',  ( 29.29714726640905909, -275.1554194970757976, -300.5582328177343356 ) ) ;
#39979=CARTESIAN_POINT ( 'NONE',  ( 34.93271569847851055, -274.3102733244279534, -258.0131353880378811 ) ) ;
#39980=CARTESIAN_POINT ( 'NONE',  ( -113.0774333050036518, -296.2294148263135298, -256.8102647436851953 ) ) ;
#39981=CARTESIAN_POINT ( 'NONE',  ( -29.40099482351953597, -125.5565301473652653, -361.1960649407547521 ) ) ;
#39982=CARTESIAN_POINT ( 'NONE',  ( 7.935645567813509160, -275.1330490791634134, -332.0972777557471431 ) ) ;
#39983=CARTESIAN_POINT ( 'NONE',  ( -81.69594748424621855, -275.1994334023129909, -211.0458463439749721 ) ) ;
#39984=CARTESIAN_POINT ( 'NONE',  ( -73.81004576435181264, -274.6595910587539606, -202.8368858384544637 ) ) ;
#39985=CARTESIAN_POINT ( 'NONE',  ( -94.14817941614803942, -290.3951673907260442, -316.3068724411707535 ) ) ;
#39986=CARTESIAN_POINT ( 'NONE',  ( -113.7815417226453434, -297.2570117141732453, -278.1783705180720858 ) ) ;
#39987=CARTESIAN_POINT ( 'NONE',  ( -78.17511752514417367, -298.0109342361442941, -205.1525378198847989 ) ) ;
#39988=CARTESIAN_POINT ( 'NONE',  ( 16.16058330017424538, -294.4326508754061820, -320.0250452585168546 ) ) ;
#39991=CARTESIAN_POINT ( 'NONE',  ( -105.0440616761899406, -280.0315030321415861, -304.0302800101594585 ) ) ;
#39992=CARTESIAN_POINT ( 'NONE',  ( -4.964175337356663498, -279.9747947529875773, -200.5669721539795489 ) ) ;
#39993=CARTESIAN_POINT ( 'NONE',  ( -6.165610532423705159, -277.5733958302975566, -336.6430231450327710 ) ) ;
#39994=CARTESIAN_POINT ( 'NONE',  ( 36.61092157524898028, -277.5342610683098314, -287.8810195974373300 ) ) ;
#39995=CARTESIAN_POINT ( 'NONE',  ( -31.60127331474626899, -275.0002645543697781, -345.5488556988973414 ) ) ;
#39996=CARTESIAN_POINT ( 'NONE',  ( -92.06841172516563176, -273.7354706260273929, -221.9568260288448869 ) ) ;
#39997=CARTESIAN_POINT ( 'NONE',  ( -65.78382479129551541, -296.2473607405311782, -202.4905023772381867 ) ) ;
#39999=CARTESIAN_POINT ( 'NONE',  ( -71.65230676159261236, -277.6854781189082360, -334.8095427585091670 ) ) ;
#40001=CARTESIAN_POINT ( 'NONE',  ( 31.23789265634772150, -286.6769697346300063, -304.3942256849774139 ) ) ;
#40002=CARTESIAN_POINT ( 'NONE',  ( -54.89100213468034895, -275.8266867059796823, -197.4432008104436136 ) ) ;
#40005=CARTESIAN_POINT ( 'NONE',  ( -86.84614854937542816, -288.9589621501868919, -324.2992449736664753 ) ) ;
#40006=CARTESIAN_POINT ( 'NONE',  ( -112.2585427403858915, -284.1179303563596932, -253.0181228491142349 ) ) ;
#40007=CARTESIAN_POINT ( 'NONE',  ( 36.53264934074726966, -279.7330155334875030, -265.8274106709538955 ) ) ;
#40008=CARTESIAN_POINT ( 'NONE',  ( 35.28215392580813869, -280.2823464980983772, -282.2418056774371280 ) ) ;
#40009=CARTESIAN_POINT ( 'NONE',  ( -38.62569617740881966, -284.1158090869892590, -195.9194602071358133 ) ) ;
#40010=CARTESIAN_POINT ( 'NONE',  ( 34.54820075568754589, -289.8281575918870203, -291.7793293692994325 ) ) ;
#40011=CARTESIAN_POINT ( 'NONE',  ( -108.8697823169071626, -279.5405664881534449, -286.8747125391779491 ) ) ;
#40013=CARTESIAN_POINT ( 'NONE',  ( -50.24789740371854663, -293.8875607099926697, -196.4799247197483965 ) ) ;
#40014=CARTESIAN_POINT ( 'NONE',  ( -113.3635260201611885, -276.8126404626281101, -268.7332873345537791 ) ) ;
#40015=CARTESIAN_POINT ( 'NONE',  ( 16.61198336187223035, -276.9103012581261964, -319.7041527892966997 ) ) ;
#40016=CARTESIAN_POINT ( 'NONE',  ( -110.7294915276277010, -286.3440450689752765, -286.6172092936743070 ) ) ;
#40017=FACE_OUTER_BOUND ( 'NONE', #40177, .T. ) ;
#40018=CARTESIAN_POINT ( 'NONE',  ( -54.15690983343117892, -291.1864617378162166, -344.0800113258711690 ) ) ;
#40019=CARTESIAN_POINT ( 'NONE',  ( -93.30674143646977825, -293.8563470380150306, -320.3657480697832511 ) ) ;
#40021=CARTESIAN_POINT ( 'NONE',  ( -26.63347344892401480, -285.3821013558943491, -194.2190146525946091 ) ) ;
#40022=CARTESIAN_POINT ( 'NONE',  ( -97.40066215283101769, -289.5457846169106801, -227.3869316750085545 ) ) ;
#40024=CARTESIAN_POINT ( 'NONE',  ( -4.863123912941094140, -275.3001110874826054, -336.3022241359696523 ) ) ;
#40025=CARTESIAN_POINT ( 'NONE',  ( -37.01348553373327377, -293.1875517288375477, -344.6082301598522690 ) ) ;
#40026=FACE_OUTER_BOUND ( 'NONE', #17293, .T. ) ;
#40027=CARTESIAN_POINT ( 'NONE',  ( -22.31123950296460379, -290.7210068484206431, -195.4955616898351707 ) ) ;
#40028=CARTESIAN_POINT ( 'NONE',  ( -94.75714959288885098, -286.8010729087941399, -223.9739966762575136 ) ) ;
#40029=CARTESIAN_POINT ( 'NONE',  ( 9.584321126841764737, -286.6569690972931426, -330.1936042499539781 ) ) ;
#40030=CARTESIAN_POINT ( 'NONE',  ( -77.38479068328094002, -286.9291271721886005, -208.5598538230038628 ) ) ;
#40033=CARTESIAN_POINT ( 'NONE',  ( -38.63800055468101391, -286.8383551428286182, -197.1986168144262592 ) ) ;
#40034=CARTESIAN_POINT ( 'NONE',  ( 37.86253805835301023, -295.6027371407022883, -275.8927440713060832 ) ) ;
#40035=CARTESIAN_POINT ( 'NONE',  ( -94.14471879594898951, -275.9449207122509051, -320.1881314391042110 ) ) ;
#40036=CARTESIAN_POINT ( 'NONE',  ( 34.16619138577753034, -276.2487381832852975, -299.0068814999503957 ) ) ;
#40037=CARTESIAN_POINT ( 'NONE',  ( -71.49901856070748352, -289.6844723970174300, -202.9480414160184978 ) ) ;
#40038=CARTESIAN_POINT ( 'NONE',  ( -108.5126566038881322, -278.9256751619376473, -240.9724304596572608 ) ) ;
#40039=CARTESIAN_POINT ( 'NONE',  ( -91.25083380922150411, -299.2613291753639260, -218.6571652577696057 ) ) ;
#40042=CARTESIAN_POINT ( 'NONE',  ( -100.2339573658729250, -276.1550768808709222, -309.8961176989543560 ) ) ;
#40043=CARTESIAN_POINT ( 'NONE',  ( 36.29599654916341223, -279.3692829281176842, -256.1312100543079850 ) ) ;
#40045=CARTESIAN_POINT ( 'NONE',  ( 3.117325199323299323, -274.9995362870396320, -335.1208733944317828 ) ) ;
#40046=CARTESIAN_POINT ( 'NONE',  ( -86.94248631422881601, -297.2778366144847837, -324.8631340983842506 ) ) ;
#40047=CARTESIAN_POINT ( 'NONE',  ( 26.45707897364511041, -281.0349414596341830, -312.9194108852886984 ) ) ;
#40048=CARTESIAN_POINT ( 'NONE',  ( -109.3713788792648813, -297.3184795589700116, -283.6643407293334462 ) ) ;
#40049=CARTESIAN_POINT ( 'NONE',  ( -101.9092417073094197, -298.4086930955334651, -229.3205180033799309 ) ) ;
#40050=CARTESIAN_POINT ( 'NONE',  ( -4.091270186654704766, -274.1698896770649867, -205.3355709942789247 ) ) ;
#40051=CARTESIAN_POINT ( 'NONE',  ( 21.74316944361589066, -294.9182611452085325, -224.1453261717357179 ) ) ;
#40052=CARTESIAN_POINT ( 'NONE',  ( 24.70201101716289571, -287.1130874018446661, -224.7587286608693091 ) ) ;
#40053=CARTESIAN_POINT ( 'NONE',  ( 34.87795658004070276, -273.9843290321488212, -293.2658481795883176 ) ) ;
#40055=CARTESIAN_POINT ( 'NONE',  ( -17.72637478188769578, -288.6392367472355431, -344.8207648797098841 ) ) ;
#40056=CARTESIAN_POINT ( 'NONE',  ( 35.50967673622771770, -286.5124201141092612, -262.8721035741455125 ) ) ;
#40057=CARTESIAN_POINT ( 'NONE',  ( -61.03204588874937286, -289.7446191059484022, -199.1462678954401895 ) ) ;
#40059=CARTESIAN_POINT ( 'NONE',  ( -28.16072294498304274, -126.4832272301380556, -368.1402060870429409 ) ) ;
#40060=CARTESIAN_POINT ( 'NONE',  ( -72.39388981885420549, -289.0370685149600263, -334.4651930453189266 ) ) ;
#40061=CARTESIAN_POINT ( 'NONE',  ( -113.5873327694909420, -285.6052001264109208, -261.4491195654939588 ) ) ;
#40062=CARTESIAN_POINT ( 'NONE',  ( 38.09624213391255410, -292.4326381615786090, -256.1506612417577458 ) ) ;
#40063=CARTESIAN_POINT ( 'NONE',  ( 12.45383555886490434, -282.3326653276039906, -212.6823087093894173 ) ) ;
#40064=CARTESIAN_POINT ( 'NONE',  ( 37.19323330833030639, -282.6494379105075723, -253.0455154827602087 ) ) ;
#40065=CARTESIAN_POINT ( 'NONE',  ( -93.42343300352005997, -283.7223755569215200, -317.0926837836212826 ) ) ;
#40066=CARTESIAN_POINT ( 'NONE',  ( 32.14024677237936345, -277.9220439890176522, -298.7352100012137726 ) ) ;
#40067=CARTESIAN_POINT ( 'NONE',  ( -108.3750413894235436, -296.1725969528496876, -300.2188811053798077 ) ) ;
#40068=CARTESIAN_POINT ( 'NONE',  ( -109.0195591655429297, -274.0800385051354624, -254.1275723580045280 ) ) ;
#40069=CARTESIAN_POINT ( 'NONE',  ( -111.4249662102223510, -288.4543579125047472, -279.4998535989397510 ) ) ;
#40071=CARTESIAN_POINT ( 'NONE',  ( -101.0548689193594072, -271.8448885987381800, -233.8204735609783995 ) ) ;
#40074=CARTESIAN_POINT ( 'NONE',  ( -107.9050110815833392, -286.7830395481826713, -246.4902024312568756 ) ) ;
#40075=CARTESIAN_POINT ( 'NONE',  ( 13.20247590706343388, -295.4448738187893468, -328.1097753205187928 ) ) ;
#40076=CARTESIAN_POINT ( 'NONE',  ( -104.2031909254667852, -284.8063894256897015, -299.9150300112569312 ) ) ;
#40077=CARTESIAN_POINT ( 'NONE',  ( 39.32012050874717346, -274.5495035605681551, -265.4667616949154194 ) ) ;
#40078=CARTESIAN_POINT ( 'NONE',  ( -92.74441215752203505, -291.9352384738761543, -216.9575723052588216 ) ) ;
#40079=CARTESIAN_POINT ( 'NONE',  ( -101.4603330445561369, -283.2289184265076187, -229.9989278496601059 ) ) ;
#40080=CARTESIAN_POINT ( 'NONE',  ( -68.32414956125494143, -291.9894821483059104, -199.8780940707751768 ) ) ;
#40081=CARTESIAN_POINT ( 'NONE',  ( -106.9709706704877163, -290.5919344085515377, -292.5249666946191383 ) ) ;
#40084=CARTESIAN_POINT ( 'NONE',  ( -38.65064075601802074, -140.2996819125500565, -360.9686471963671011 ) ) ;
#40085=CARTESIAN_POINT ( 'NONE',  ( -16.31414505355634859, -284.3054154541990783, -343.7681407864705534 ) ) ;
#40086=CARTESIAN_POINT ( 'NONE',  ( -37.37352853689063181, -292.5523547857347353, -345.3611179825600175 ) ) ;
#40089=CARTESIAN_POINT ( 'NONE',  ( 5.762795176377190742, -281.3725869330493765, -329.6589135343029966 ) ) ;
#40090=CARTESIAN_POINT ( 'NONE',  ( -48.49511986439432576, -276.8570119589404044, -346.5815622534594809 ) ) ;
#40091=CARTESIAN_POINT ( 'NONE',  ( -103.7953643696253891, -281.0100932169717680, -235.8398544096079377 ) ) ;
#40092=CARTESIAN_POINT ( 'NONE',  ( -61.32887853807750389, -183.8452602080190559, -360.6299234569646615 ) ) ;
#40093=CARTESIAN_POINT ( 'NONE',  ( -13.62220642536452431, -281.3248584795038028, -342.9971414855608600 ) ) ;
#40094=CARTESIAN_POINT ( 'NONE',  ( -108.9252590724021985, -282.8481418639596541, -249.0245356062137319 ) ) ;
#40095=CARTESIAN_POINT ( 'NONE',  ( -15.20086602440459167, -300.0858634728058405, -194.3679151187695027 ) ) ;
#40096=CARTESIAN_POINT ( 'NONE',  ( -94.81796891096114166, -296.4089913983243036, -315.4661838695809024 ) ) ;
#40098=CARTESIAN_POINT ( 'NONE',  ( 26.67228065799706371, -291.7448882022110865, -234.1537904275760127 ) ) ;
#40099=CARTESIAN_POINT ( 'NONE',  ( 39.27963928983869835, -276.2851872958053150, -276.8790265555686005 ) ) ;
#40100=CARTESIAN_POINT ( 'NONE',  ( 35.37821433383642500, -275.4605971271983549, -263.4207455564619522 ) ) ;
#40101=CARTESIAN_POINT ( 'NONE',  ( 9.333141660948436780, -273.5971488577953323, -209.5092350794786569 ) ) ;
#40103=CARTESIAN_POINT ( 'NONE',  ( -64.66280059341735864, -271.6953017060425282, -200.5007660474314832 ) ) ;
#40107=CARTESIAN_POINT ( 'NONE',  ( 33.26084032723394301, -282.8915765668057247, -290.0970586854664930 ) ) ;
#40108=CARTESIAN_POINT ( 'NONE',  ( 0.3849813559168659971, -284.3169310994955481, -336.3357722944173247 ) ) ;
#40109=CARTESIAN_POINT ( 'NONE',  ( -106.2726213801001620, -283.5754797676106023, -294.8516004122698746 ) ) ;
#40110=CARTESIAN_POINT ( 'NONE',  ( 5.848655634099327649, -274.8559055013023453, -330.2659502610648019 ) ) ;
#40111=CARTESIAN_POINT ( 'NONE',  ( -18.39794291737094412, -284.6660543387716871, -342.1918443868438544 ) ) ;
#40112=CARTESIAN_POINT ( 'NONE',  ( -109.7279446866395318, -276.8505860660528697, -284.2459637580699905 ) ) ;
#40113=CARTESIAN_POINT ( 'NONE',  ( 35.01451377247138907, -276.7906239789874689, -282.4497198349457676 ) ) ;
#40115=CARTESIAN_POINT ( 'NONE',  ( -104.6570544767593276, -279.8358793108898794, -233.3097767252989740 ) ) ;
#40118=CYLINDRICAL_SURFACE ( 'NONE', #32287, 6.154241149514405151 ) ;
#40119=CARTESIAN_POINT ( 'NONE',  ( -69.29385972965550877, -287.4967074610819964, -201.6493469937357474 ) ) ;
#40120=CARTESIAN_POINT ( 'NONE',  ( -9.178148466532000782, -293.8714332438996735, -337.8982013936831663 ) ) ;
#40121=CARTESIAN_POINT ( 'NONE',  ( -109.3754374719327984, -290.2433117206783209, -243.2937418133845142 ) ) ;
#40122=CARTESIAN_POINT ( 'NONE',  ( 35.51529902032152819, -285.9615671557526753, -283.3930668013445029 ) ) ;
#40123=CARTESIAN_POINT ( 'NONE',  ( 32.84097504660392275, -285.8353667372550717, -248.1882171182276977 ) ) ;
#40124=CARTESIAN_POINT ( 'NONE',  ( -110.6294709175320889, -288.6563108310282360, -280.7903528653516219 ) ) ;
#40125=CARTESIAN_POINT ( 'NONE',  ( -61.65184179818690779, -284.5801319743679869, -339.6688627353864263 ) ) ;
#40126=CARTESIAN_POINT ( 'NONE',  ( 36.94675294573447388, -273.4196546582299447, -260.0544993018278319 ) ) ;
#40127=CARTESIAN_POINT ( 'NONE',  ( -0.08932612986281238121, -284.9390668879638611, -203.8729140247605756 ) ) ;
#40128=CARTESIAN_POINT ( 'NONE',  ( -69.88487936619216612, -299.6237110299645110, -202.7893625008937022 ) ) ;
#40129=CARTESIAN_POINT ( 'NONE',  ( 18.25075829543008155, -286.2565682532813298, -320.9718525808416416 ) ) ;
#40130=CARTESIAN_POINT ( 'NONE',  ( 33.68083679361920701, -282.2577693448175751, -252.4438174280260228 ) ) ;
#40131=CARTESIAN_POINT ( 'NONE',  ( -69.82321471852675643, -291.4789367081937144, -338.1615362372652385 ) ) ;
#40134=CARTESIAN_POINT ( 'NONE',  ( -37.65794076881845598, -296.9761954410017211, -345.9332944128814233 ) ) ;
#40136=CARTESIAN_POINT ( 'NONE',  ( -32.81760037415347853, -278.1090144348538615, -195.4976878484475264 ) ) ;
#40137=CARTESIAN_POINT ( 'NONE',  ( -69.54613633110318460, -290.8361624137102694, -200.5826824542176041 ) ) ;
#40138=CARTESIAN_POINT ( 'NONE',  ( -96.25513867432701431, -294.3341962493550454, -314.8301954895704853 ) ) ;
#40139=CARTESIAN_POINT ( 'NONE',  ( 5.868614539845057543, -281.1371222281718474, -329.8095173136823064 ) ) ;
#40140=CARTESIAN_POINT ( 'NONE',  ( 3.744721200102505421, -272.6892301998387893, -208.2251898951031137 ) ) ;
#40141=CARTESIAN_POINT ( 'NONE',  ( 36.11369905372555422, -294.8364704761917210, -268.0057395224523020 ) ) ;
#40142=CARTESIAN_POINT ( 'NONE',  ( -110.4542110544635705, -286.8376638359844719, -287.0812184334320705 ) ) ;
#40143=CARTESIAN_POINT ( 'NONE',  ( -111.3014765373895472, -294.7943154103827510, -289.1931454069718370 ) ) ;
#40144=CARTESIAN_POINT ( 'NONE',  ( 38.59341007484657382, -291.8274801446793276, -273.1598766159764295 ) ) ;
#40145=CARTESIAN_POINT ( 'NONE',  ( -65.56963253740221376, -293.1009461683775044, -202.3875140202095508 ) ) ;
#40147=CARTESIAN_POINT ( 'NONE',  ( 21.11667801393515731, -293.7385796721616202, -226.3699853258602559 ) ) ;
#40149=CARTESIAN_POINT ( 'NONE',  ( -93.19729783831272130, -281.8700073868677691, -320.9624640002090246 ) ) ;
#40150=CARTESIAN_POINT ( 'NONE',  ( -66.05313749947666224, -295.4386775450634559, -337.4778324735751767 ) ) ;
#40151=CARTESIAN_POINT ( 'NONE',  ( 38.66784513340837748, -281.7071423286387812, -282.7540055199416429 ) ) ;
#40152=CARTESIAN_POINT ( 'NONE',  ( -66.57215317191126758, -283.0913821453785317, -341.5885358424188780 ) ) ;
#40153=CARTESIAN_POINT ( 'NONE',  ( -42.82300483389046519, -287.1211847448572030, -345.0453166641094072 ) ) ;
#40155=CARTESIAN_POINT ( 'NONE',  ( 31.75626198119757504, -280.4517813083118085, -302.8611370630159740 ) ) ;
#40156=CARTESIAN_POINT ( 'NONE',  ( 36.48310307912309014, -286.7343657243646931, -291.1791992913473450 ) ) ;
#40158=CARTESIAN_POINT ( 'NONE',  ( -47.88742736761130914, -296.7884936568450485, -343.4556035799229221 ) ) ;
#40159=CARTESIAN_POINT ( 'NONE',  ( -73.79961244147870048, -278.9517256555167251, -337.5282702082107562 ) ) ;
#40160=CARTESIAN_POINT ( 'NONE',  ( -62.31219064049827949, -279.3850568356900794, -201.6887835738847343 ) ) ;
#40161=CARTESIAN_POINT ( 'NONE',  ( -37.79715997090553969, -292.2132741407780827, -193.3624650016934368 ) ) ;
#40162=CARTESIAN_POINT ( 'NONE',  ( -6.074148943219241481, -280.7242895402707177, -339.1481403360583045 ) ) ;
#40163=CARTESIAN_POINT ( 'NONE',  ( -12.16810478285903940, -291.4465099774787404, -201.5342592106387087 ) ) ;
#40165=CARTESIAN_POINT ( 'NONE',  ( -88.23203679673940769, -295.3398691553587696, -215.1983737472510256 ) ) ;
#40167=CARTESIAN_POINT ( 'NONE',  ( -37.00155433637099378, -294.5553988545158290, -343.4342994320877551 ) ) ;
#40169=CARTESIAN_POINT ( 'NONE',  ( -102.0172624299487154, -288.4809262143061801, -239.1787733560258289 ) ) ;
#40170=CARTESIAN_POINT ( 'NONE',  ( -35.82186107926352037, -297.1294972969841410, -193.5966463115552187 ) ) ;
#40171=CARTESIAN_POINT ( 'NONE',  ( 26.81817931088598073, -279.1544078907135713, -229.9661576509479062 ) ) ;
#40172=CARTESIAN_POINT ( 'NONE',  ( -3.721273210295284350, -287.8016481334057630, -201.6228523707503371 ) ) ;
#40173=CARTESIAN_POINT ( 'NONE',  ( 21.17221221186893487, -287.9981436606121861, -314.0297462076907777 ) ) ;
#40174=CARTESIAN_POINT ( 'NONE',  ( -91.46401832657168995, -279.3599840078262559, -320.4501432748168099 ) ) ;
#40175=CARTESIAN_POINT ( 'NONE',  ( -60.85882815576348293, -299.5030410351093906, -200.1291356229187386 ) ) ;
#40176=CARTESIAN_POINT ( 'NONE',  ( -99.51959407465871266, -276.8103114638750526, -309.4565968598176937 ) ) ;
#40177=EDGE_LOOP ( 'NONE', ( #25118, #75403 ) ) ;
#40178=CARTESIAN_POINT ( 'NONE',  ( 7.977900039700807966, -298.2717498065657082, -193.3847308610179709 ) ) ;
#40179=CARTESIAN_POINT ( 'NONE',  ( -105.3536124538997711, -292.0713083396632328, -300.7487589939452164 ) ) ;
#40180=CARTESIAN_POINT ( 'NONE',  ( 31.51594013473109257, -295.5762779928133455, -303.1195342151915497 ) ) ;
#40181=CARTESIAN_POINT ( 'NONE',  ( -112.3417001281054297, -274.5519904173220311, -270.3865538441530134 ) ) ;
#40182=CARTESIAN_POINT ( 'NONE',  ( -84.74483085874628330, -290.3770266918165248, -326.0771471112191762 ) ) ;
#40184=EDGE_LOOP ( 'NONE', ( #87033, #73988, #57834, #60165, #59226 ) ) ;
#40185=CARTESIAN_POINT ( 'NONE',  ( -108.2777975997807687, -296.8239053091572259, -300.1869908493025036 ) ) ;
#40186=CARTESIAN_POINT ( 'NONE',  ( -102.7443338610062398, -288.1846738122455918, -308.7115243331081160 ) ) ;
#40187=CARTESIAN_POINT ( 'NONE',  ( -20.51992406059540386, -298.5906499936787668, -193.3813386032300627 ) ) ;
#40190=CARTESIAN_POINT ( 'NONE',  ( -92.32605091355844706, -292.8038071451268820, -217.3762944957956904 ) ) ;
#40191=CARTESIAN_POINT ( 'NONE',  ( -115.3288506153726871, -292.8376638359844719, -288.1938231032136741 ) ) ;
#40193=CARTESIAN_POINT ( 'NONE',  ( -112.1426021787407734, -286.5806676322059730, -268.1580574037957945 ) ) ;
#40194=EDGE_CURVE ( 'NONE', #64758, #52349, #22824, .T. ) ;
#40195=CARTESIAN_POINT ( 'NONE',  ( -35.31579140500846847, -272.0774514714984775, -195.5423891952795259 ) ) ;
#40196=CARTESIAN_POINT ( 'NONE',  ( -94.02589681328788629, -275.1454823192548815, -222.0898422885150012 ) ) ;
#40197=CARTESIAN_POINT ( 'NONE',  ( -88.91088281404442739, -289.4011311945246234, -216.6062619644874587 ) ) ;
#40198=CARTESIAN_POINT ( 'NONE',  ( -111.5132822861773860, -280.6098023860867556, -254.8426522913349572 ) ) ;
#40200=CARTESIAN_POINT ( 'NONE',  ( -32.96301398965226781, -280.1088519242433676, -197.4925574938202431 ) ) ;
#40201=CARTESIAN_POINT ( 'NONE',  ( 13.41183382841328786, -280.1336181705341914, -217.6790537174373128 ) ) ;
#40202=CARTESIAN_POINT ( 'NONE',  ( -1.599553540020983267, -277.6692916526148451, -338.2138369244971159 ) ) ;
#40203=CARTESIAN_POINT ( 'NONE',  ( -36.74017999978996585, -278.8544850417941348, -193.7475722532458633 ) ) ;
#40204=CARTESIAN_POINT ( 'NONE',  ( 24.07068301800163468, -23.09745244138832021, -342.0737546775265514 ) ) ;
#40205=CARTESIAN_POINT ( 'NONE',  ( 11.62635313455881558, -275.6535988416750342, -211.1739514600166103 ) ) ;
#40207=CARTESIAN_POINT ( 'NONE',  ( -93.64686790491953161, -274.7792567582446281, -218.8400156709825524 ) ) ;
#40208=CARTESIAN_POINT ( 'NONE',  ( -106.6379572354042296, -298.6233781216988632, -303.7686719486574702 ) ) ;
#40211=CARTESIAN_POINT ( 'NONE',  ( 32.12915457211946091, -288.3221465360573461, -246.9511538494989793 ) ) ;
#40212=CARTESIAN_POINT ( 'NONE',  ( 17.92341329464438715, -290.0339282662094433, -322.5122565315427892 ) ) ;
#40213=CARTESIAN_POINT ( 'NONE',  ( -72.41504633432106175, -288.8780281951142115, -334.4996637586543784 ) ) ;
#40214=CARTESIAN_POINT ( 'NONE',  ( 5.150917078162668084, -286.1174522227927355, -206.1579332821879404 ) ) ;
#40216=CARTESIAN_POINT ( 'NONE',  ( 16.39453744152071479, -280.6730977097220716, -321.0199702973334297 ) ) ;
#40217=CARTESIAN_POINT ( 'NONE',  ( -20.83197491482815167, -290.6984114718369483, -342.7371806746199354 ) ) ;
#40218=CARTESIAN_POINT ( 'NONE',  ( -93.09625896302375736, -282.3517350958592260, -318.5688835727382866 ) ) ;
#40219=CARTESIAN_POINT ( 'NONE',  ( -41.09299418832080875, -281.3191294910885176, -196.9637660435205930 ) ) ;
#40220=CARTESIAN_POINT ( 'NONE',  ( -5.033232194831216866, -277.1073396884305566, -335.9047950491271308 ) ) ;
#40221=CARTESIAN_POINT ( 'NONE',  ( -99.55679244840483477, -288.7514205678791654, -315.0746592334719480 ) ) ;
#40222=CARTESIAN_POINT ( 'NONE',  ( -113.3293070806293059, -285.5023006148979903, -258.6063387006830112 ) ) ;
#40223=CARTESIAN_POINT ( 'NONE',  ( -63.18666872767307296, -286.2166709612661180, -197.8934389715013822 ) ) ;
#40224=CARTESIAN_POINT ( 'NONE',  ( 35.03250150065544233, -281.5880532896999284, -260.4472952927281426 ) ) ;
#40225=ORIENTED_EDGE ( 'NONE', *, *, #17187, .T. ) ;
#40227=CARTESIAN_POINT ( 'NONE',  ( -91.93870168046433378, -293.1440462414617514, -217.7557679270126982 ) ) ;
#40229=CARTESIAN_POINT ( 'NONE',  ( -37.77532100652363312, -290.7316599778227442, -193.8554956534819951 ) ) ;
#40230=CARTESIAN_POINT ( 'NONE',  ( 25.48382586996844523, -274.0937351059172329, -232.6282847950508597 ) ) ;
#40231=CARTESIAN_POINT ( 'NONE',  ( -74.56430276819779124, -294.8821865711833539, -337.7096142731411419 ) ) ;
#40232=CARTESIAN_POINT ( 'NONE',  ( -86.37606391125603977, -289.8369702536953696, -215.2802791846533523 ) ) ;
#40233=CARTESIAN_POINT ( 'NONE',  ( -34.28142380136883816, -293.2530057701960686, -344.3111600648140325 ) ) ;
#40234=CARTESIAN_POINT ( 'NONE',  ( -70.13614598002813239, -290.6992528245734775, -336.0382429879452957 ) ) ;
#40236=CARTESIAN_POINT ( 'NONE',  ( -64.69327756281664676, -291.4093006799419641, -340.2507352403997629 ) ) ;
#40237=CARTESIAN_POINT ( 'NONE',  ( 24.98730492991275653, -290.9838813684707475, -228.2561406114209888 ) ) ;
#40238=CARTESIAN_POINT ( 'NONE',  ( -7.211395784144283283, -296.6572533313993176, -339.0974399810747855 ) ) ;
#40239=CARTESIAN_POINT ( 'NONE',  ( -2.083597929016404837, -287.4720173169050099, -206.1148572225795874 ) ) ;
#40240=CARTESIAN_POINT ( 'NONE',  ( -4.564827007459695274, -276.4616969223038723, -202.4935258645224394 ) ) ;
#40241=CARTESIAN_POINT ( 'NONE',  ( -70.14498173764704347, -276.2696582441936357, -339.5994189165526222 ) ) ;
#40242=CARTESIAN_POINT ( 'NONE',  ( -78.10811599370715896, -296.7159632423421840, -205.2284982153708199 ) ) ;
#40243=CARTESIAN_POINT ( 'NONE',  ( 33.86674326999936113, -274.0557201147880733, -290.5899046316356475 ) ) ;
#40244=CARTESIAN_POINT ( 'NONE',  ( -96.74641479322900750, -277.2502375335812417, -225.4802528007515434 ) ) ;
#40245=CARTESIAN_POINT ( 'NONE',  ( -43.53082439929039538, -275.1774514536521679, -197.1744677493692848 ) ) ;
#40246=CARTESIAN_POINT ( 'NONE',  ( -4.359748912820315958, -275.0245934224437860, -339.0677583208797614 ) ) ;
#40248=CARTESIAN_POINT ( 'NONE',  ( -100.8103800471136680, -273.7010786471676624, -233.9878389500318008 ) ) ;
#40250=CARTESIAN_POINT ( 'NONE',  ( -73.65725780624509866, -287.5517500862881093, -336.4030215070834515 ) ) ;
#40251=CARTESIAN_POINT ( 'NONE',  ( 7.332587685620199913, -274.5142294574891366, -212.6271763812662527 ) ) ;
#40252=CARTESIAN_POINT ( 'NONE',  ( -28.97717893952974322, -288.9490459424088726, -346.9589760704899390 ) ) ;
#40253=CARTESIAN_POINT ( 'NONE',  ( -62.76067725732410452, -289.0407487716310015, -343.0784809513011169 ) ) ;
#40254=CARTESIAN_POINT ( 'NONE',  ( -96.38909544602353208, -275.1895370155652927, -223.8483935142291443 ) ) ;
#40255=CARTESIAN_POINT ( 'NONE',  ( -42.54192650756851890, -293.1177497468139563, -345.0135531265428881 ) ) ;
#40256=CARTESIAN_POINT ( 'NONE',  ( 39.36726158846801837, -280.8157299222871188, -275.6599710469711226 ) ) ;
#40258=CARTESIAN_POINT ( 'NONE',  ( -111.7861933247250050, -276.4297109563016761, -279.8844756648734347 ) ) ;
#40260=CARTESIAN_POINT ( 'NONE',  ( -98.44972449581582907, -288.7855000624626882, -311.0403685920500152 ) ) ;
#40262=CARTESIAN_POINT ( 'NONE',  ( -105.3597193119151711, -288.9671867823670368, -238.7612807683443634 ) ) ;
#40263=CARTESIAN_POINT ( 'NONE',  ( -2.603770651260073343, -276.0405163377008648, -205.3689337651601932 ) ) ;
#40264=CARTESIAN_POINT ( 'NONE',  ( 37.40445599313808600, -282.7767182098007197, -254.4361061248319231 ) ) ;
#40265=CARTESIAN_POINT ( 'NONE',  ( -37.57667570481402919, -296.0693364529760743, -195.0062800877014979 ) ) ;
#40266=CARTESIAN_POINT ( 'NONE',  ( -58.94813133534841398, -283.3394758848206720, -340.1434654586647639 ) ) ;
#40267=CARTESIAN_POINT ( 'NONE',  ( -36.74941432824717680, -275.4850115414347442, -196.7617556734629716 ) ) ;
#40268=CARTESIAN_POINT ( 'NONE',  ( -8.917513416117403224, -275.2364175145195304, -202.8929433299195466 ) ) ;
#40269=CARTESIAN_POINT ( 'NONE',  ( 36.69238179845905989, -285.8245570761948784, -285.4696888794601364 ) ) ;
#40270=CARTESIAN_POINT ( 'NONE',  ( 25.07202786556470286, -284.1142764794475966, -311.9487027491192066 ) ) ;
#40271=CARTESIAN_POINT ( 'NONE',  ( 9.128316012624253517, -297.7066625357991825, -197.1334806806277129 ) ) ;
#40274=CARTESIAN_POINT ( 'NONE',  ( -16.50891973755927822, -294.6236239495773361, -344.5445855467741580 ) ) ;
#40275=CARTESIAN_POINT ( 'NONE',  ( -103.2110607073295370, -286.0627493961774803, -305.5862152029044978 ) ) ;
#40277=CARTESIAN_POINT ( 'NONE',  ( -72.02372285203398405, -271.1237833571632905, -198.2697987213421698 ) ) ;
#40278=CARTESIAN_POINT ( 'NONE',  ( -74.02876733551443067, -276.7239807225424215, -337.8906650403386038 ) ) ;
#40279=CARTESIAN_POINT ( 'NONE',  ( -112.8703660387259760, -289.0844462595420623, -259.8829617893832733 ) ) ;
#40280=CARTESIAN_POINT ( 'NONE',  ( -3.283904601745656571, -284.1140271832124427, -335.7264192126351645 ) ) ;
#40281=CARTESIAN_POINT ( 'NONE',  ( -32.32985693659846049, -278.7483780957962267, -344.2552296789129969 ) ) ;
#40282=CARTESIAN_POINT ( 'NONE',  ( -109.4274434302726320, -286.2995768828680525, -245.0184286087743715 ) ) ;
#40283=CARTESIAN_POINT ( 'NONE',  ( 1.412156205598005698, -282.5696769494897467, -206.0893352650113570 ) ) ;
#40284=CARTESIAN_POINT ( 'NONE',  ( 7.233260528640313325, -274.8074478649547245, -207.5097556160975500 ) ) ;
#40285=CARTESIAN_POINT ( 'NONE',  ( -67.71056107890268549, -277.2731252454187825, -341.1193845601805492 ) ) ;
#40286=CARTESIAN_POINT ( 'NONE',  ( -70.34085681697077064, -297.4107243580212412, -337.0871987860103332 ) ) ;
#40290=CARTESIAN_POINT ( 'NONE',  ( -113.1681449034579288, -270.8640168928444609, -264.6793891393130025 ) ) ;
#40291=CARTESIAN_POINT ( 'NONE',  ( 35.66308864001567969, -275.1120112299278162, -274.3222119941613073 ) ) ;
#40292=CARTESIAN_POINT ( 'NONE',  ( -43.27959702465449254, -299.0586335826179720, -193.8474522296141913 ) ) ;
#40293=CARTESIAN_POINT ( 'NONE',  ( -49.61128450112837385, -287.6538493211135119, -197.3196473749968902 ) ) ;
#40294=CARTESIAN_POINT ( 'NONE',  ( -110.1325382354403928, -297.7814505541182939, -293.3002672883740161 ) ) ;
#40295=CARTESIAN_POINT ( 'NONE',  ( -113.9410608491082826, -297.7665210643149294, -269.6217570473887122 ) ) ;
#40297=CARTESIAN_POINT ( 'NONE',  ( -80.61100830522308058, -293.4645102622918102, -209.2419138053886627 ) ) ;
#40298=CARTESIAN_POINT ( 'NONE',  ( -16.38448002622649824, -278.3234877718984421, -198.5222472401431162 ) ) ;
#40299=CARTESIAN_POINT ( 'NONE',  ( -72.83746676551753296, -281.4982014040226659, -204.9289794691087536 ) ) ;
#40300=CARTESIAN_POINT ( 'NONE',  ( -63.56427577703370702, -295.7876930335344809, -200.6381576156095150 ) ) ;
#40301=CARTESIAN_POINT ( 'NONE',  ( -60.82593478213906479, -285.2139741538793487, -342.4492017140225357 ) ) ;
#40302=CARTESIAN_POINT ( 'NONE',  ( 16.20962641980324292, -285.7551229352160931, -220.2778162924574872 ) ) ;
#40303=CARTESIAN_POINT ( 'NONE',  ( -69.43587163635656623, -197.0798774606213044, -360.0883899004672344 ) ) ;
#40305=CARTESIAN_POINT ( 'NONE',  ( 32.29503628924079806, -286.9271816716953936, -248.3462560050296020 ) ) ;
#40307=CARTESIAN_POINT ( 'NONE',  ( 36.68302432211552855, -282.3792019230424444, -250.2655865881534965 ) ) ;
#40308=CARTESIAN_POINT ( 'NONE',  ( -91.14098625775427820, -273.5939946197576091, -220.9692914688024814 ) ) ;
#40309=CARTESIAN_POINT ( 'NONE',  ( 13.99223219465214463, -285.5482619160324020, -213.4319043924199946 ) ) ;
#40310=CARTESIAN_POINT ( 'NONE',  ( -22.62307397294971878, -281.1772391186856339, -194.9665872965468338 ) ) ;
#40312=CARTESIAN_POINT ( 'NONE',  ( -109.8965370368623411, -280.3741776000559867, -246.5606030017572152 ) ) ;
#40313=CARTESIAN_POINT ( 'NONE',  ( -1.149130967571978967, -280.8523583744608914, -202.4211280712816858 ) ) ;
#40314=CARTESIAN_POINT ( 'NONE',  ( -21.33282851196157992, -283.7666405000204009, -200.3683826091710216 ) ) ;
#40315=CARTESIAN_POINT ( 'NONE',  ( -30.68111782768947648, -124.5880914476725820, -364.4545987036558472 ) ) ;
#40317=CARTESIAN_POINT ( 'NONE',  ( -46.42597181955041918, -275.9367614358185961, -196.0812119987735400 ) ) ;
#40318=CARTESIAN_POINT ( 'NONE',  ( -40.31272606951220894, -139.2760872083653112, -364.4166386884767235 ) ) ;
#40319=CARTESIAN_POINT ( 'NONE',  ( 20.61347554750452815, -280.2234616458142682, -317.4242637509498763 ) ) ;
#40320=CARTESIAN_POINT ( 'NONE',  ( -30.80705249287348124, -293.8936763090558770, -194.6038864475353876 ) ) ;
#40321=CARTESIAN_POINT ( 'NONE',  ( -28.89242184229226496, -294.2909349696849404, -343.0242011832186790 ) ) ;
#40322=CARTESIAN_POINT ( 'NONE',  ( -42.04393268639119441, -291.5020270628396588, -193.5664833245303100 ) ) ;
#40324=CARTESIAN_POINT ( 'NONE',  ( -93.27065634060967625, -294.4115757982546597, -322.4434147832793087 ) ) ;
#40325=CARTESIAN_POINT ( 'NONE',  ( 31.73047897364953585, -285.6072588459414305, -244.2268595623524163 ) ) ;
#40326=CARTESIAN_POINT ( 'NONE',  ( 34.49766186445496174, -295.1696950398659283, -251.6535913892309395 ) ) ;
#40327=CARTESIAN_POINT ( 'NONE',  ( -96.17069049695247429, -286.4814759086748950, -226.3112215992280767 ) ) ;
#40329=CARTESIAN_POINT ( 'NONE',  ( 37.52914483312031990, -294.2801461510863987, -253.3559323539323884 ) ) ;
#40330=CARTESIAN_POINT ( 'NONE',  ( 30.39392505035694825, -282.4108956579887035, -297.7449366204801890 ) ) ;
#40331=CARTESIAN_POINT ( 'NONE',  ( -41.93716073505599695, -293.9036425995275863, -346.8782031763719260 ) ) ;
#40332=CARTESIAN_POINT ( 'NONE',  ( -85.05638526987864623, -290.4942147617866226, -330.6574590484464125 ) ) ;
#40333=CARTESIAN_POINT ( 'NONE',  ( -8.540078410623545224, -292.9115321787788275, -199.0169276814324633 ) ) ;
#40334=CARTESIAN_POINT ( 'NONE',  ( -18.47145725416471507, -288.9690159218346253, -340.9325948489732241 ) ) ;
#40337=CARTESIAN_POINT ( 'NONE',  ( -111.0978075727358743, -298.1915749314243271, -287.7475409260036372 ) ) ;
#40338=CARTESIAN_POINT ( 'NONE',  ( 75.49899281977172905, -298.1218452906548464, -193.8788234879655477 ) ) ;
#40339=CARTESIAN_POINT ( 'NONE',  ( -22.13388136519051130, -279.3103712974322548, -198.6702010224383059 ) ) ;
#40340=CARTESIAN_POINT ( 'NONE',  ( 34.12476320728853096, -275.4232427413429036, -299.0015947809164345 ) ) ;
#40341=CARTESIAN_POINT ( 'NONE',  ( -68.32150903723427859, -296.1175592700974448, -203.4820934126534837 ) ) ;
#40342=CARTESIAN_POINT ( 'NONE',  ( -68.53524459840360805, -279.3268666977951398, -337.7385001781133269 ) ) ;
#40343=CARTESIAN_POINT ( 'NONE',  ( 35.36970726023576361, -273.8858488169000793, -285.3249650392575063 ) ) ;
#40344=CARTESIAN_POINT ( 'NONE',  ( -99.05891737047200252, -297.2093039881702907, -310.1796985396794071 ) ) ;
#40345=CARTESIAN_POINT ( 'NONE',  ( -108.1377471099350771, -297.8826929133082899, -251.2825818296008435 ) ) ;
#40347=CARTESIAN_POINT ( 'NONE',  ( -77.79519343797886677, -299.1185368534624445, -205.7859269755718969 ) ) ;
#40348=CARTESIAN_POINT ( 'NONE',  ( -104.1390115208792650, -271.0333383620821905, -235.3696795757728353 ) ) ;
#40349=CARTESIAN_POINT ( 'NONE',  ( -69.06933624462200783, -292.2749678855324191, -204.4894953015212593 ) ) ;
#40350=CARTESIAN_POINT ( 'NONE',  ( -106.2561030079704665, -289.4701729014945499, -244.4061591369993209 ) ) ;
#40352=CARTESIAN_POINT ( 'NONE',  ( -15.80060419697402629, -274.8157711547287363, -196.4444133984104326 ) ) ;
#40353=CARTESIAN_POINT ( 'NONE',  ( -44.57540178027967670, -298.2915238935011644, -197.6487571438956365 ) ) ;
#40354=CARTESIAN_POINT ( 'NONE',  ( -71.77813887535351967, -281.5792859684895006, -203.3203762048489125 ) ) ;
#40355=CARTESIAN_POINT ( 'NONE',  ( 15.40136942118950714, -281.0100184163943595, -325.7819343458215826 ) ) ;
#40356=CARTESIAN_POINT ( 'NONE',  ( -37.13557863764886946, -276.3981907261499487, -347.2719504756964284 ) ) ;
#40357=CARTESIAN_POINT ( 'NONE',  ( -69.08846317310552365, -282.6778941922639206, -336.2896305014791096 ) ) ;
#40358=CARTESIAN_POINT ( 'NONE',  ( -4.976858644766549489, -280.6269117199074685, -338.2173220153252373 ) ) ;
#40359=CARTESIAN_POINT ( 'NONE',  ( 31.67719204698937219, -273.7891802211075856, -244.8313816107037439 ) ) ;
#40360=CARTESIAN_POINT ( 'NONE',  ( -77.09343530281887524, -279.5845995019289489, -334.0202496965131331 ) ) ;
#40363=CARTESIAN_POINT ( 'NONE',  ( -113.3811844794317523, -271.0240039671355134, -264.6655298172289577 ) ) ;
#40364=CARTESIAN_POINT ( 'NONE',  ( -111.4864747299796903, -280.3940606598785621, -282.7134791763288604 ) ) ;
#40366=CARTESIAN_POINT ( 'NONE',  ( -87.34984184609383817, -285.6628006742843695, -327.0745821107507254 ) ) ;
#40369=CARTESIAN_POINT ( 'NONE',  ( 31.75630755827969054, -285.9345024919887237, -299.6557161273402698 ) ) ;
#40371=CARTESIAN_POINT ( 'NONE',  ( -109.4327953167447873, -295.5288032931941871, -256.5100406723342985 ) ) ;
#40372=CARTESIAN_POINT ( 'NONE',  ( -10.29579733056928958, -286.8351161843877435, -339.5493368639119467 ) ) ;
#40373=CARTESIAN_POINT ( 'NONE',  ( -114.4693872376281121, -273.8646567567205921, -270.3778293100139649 ) ) ;
#40374=CARTESIAN_POINT ( 'NONE',  ( -95.13895651526389940, -295.2117323986929023, -222.5449353558778682 ) ) ;
#40375=CARTESIAN_POINT ( 'NONE',  ( -43.59001445993780521, -284.4545852699117177, -194.2579191291870302 ) ) ;
#40376=CARTESIAN_POINT ( 'NONE',  ( 11.82378249062202435, -282.3489499875647084, -215.3229881791442040 ) ) ;
#40377=CARTESIAN_POINT ( 'NONE',  ( -38.73671833641064666, -281.3092890223567224, -346.3349815211871601 ) ) ;
#40378=CARTESIAN_POINT ( 'NONE',  ( -68.75797821553327083, -289.4770535021120850, -336.2551045908377318 ) ) ;
#40379=CARTESIAN_POINT ( 'NONE',  ( -38.38026192130610781, -281.4641603985535880, -196.7667147504528771 ) ) ;
#40380=CARTESIAN_POINT ( 'NONE',  ( -67.38191867309103600, -280.4506382189260876, -203.6377586362480088 ) ) ;
#40381=CARTESIAN_POINT ( 'NONE',  ( 35.77465287620216827, -289.2989616883940016, -252.1291205649638982 ) ) ;
#40383=CARTESIAN_POINT ( 'NONE',  ( -68.84406436175810029, -273.6493352913957438, -200.0857731646960644 ) ) ;
#40384=CARTESIAN_POINT ( 'NONE',  ( -97.06960495634615427, -291.9171652815668949, -315.1532361103663789 ) ) ;
#40386=CARTESIAN_POINT ( 'NONE',  ( -2.659677404128715672, -294.9805209788416391, -198.2697987213421698 ) ) ;
#40388=CARTESIAN_POINT ( 'NONE',  ( 7.135258860325478736, -274.4481728422265405, -331.0211601069844960 ) ) ;
#40390=CARTESIAN_POINT ( 'NONE',  ( -4.862215199290253587, -293.0314558350275433, -339.3067306606041029 ) ) ;
#40391=CARTESIAN_POINT ( 'NONE',  ( -33.80207301770183648, -297.6052914145107593, -197.2998848337567495 ) ) ;
#40392=CARTESIAN_POINT ( 'NONE',  ( -48.14366626442389219, -290.7120622004322854, -343.3099846582894656 ) ) ;
#40393=CARTESIAN_POINT ( 'NONE',  ( -71.86191250414461251, -285.2751981996870541, -335.8311794829868973 ) ) ;
#40394=CARTESIAN_POINT ( 'NONE',  ( -42.03603457924297260, -293.4193369162962313, -194.0946802960376374 ) ) ;
#40395=CARTESIAN_POINT ( 'NONE',  ( -94.35506148009609717, -292.5637789856312452, -219.3437199637074571 ) ) ;
#40396=CARTESIAN_POINT ( 'NONE',  ( -55.25814271919125531, -287.8219893323475844, -197.4788053075515109 ) ) ;
#40397=CARTESIAN_POINT ( 'NONE',  ( -77.49432812584645092, -279.6961669607036924, -204.5972872974077177 ) ) ;
#40398=CARTESIAN_POINT ( 'NONE',  ( -111.7172948236253944, -294.8018386491282286, -257.0350115200009213 ) ) ;
#40399=CARTESIAN_POINT ( 'NONE',  ( -92.43521982086667776, -283.6475701645995855, -324.1542782574650232 ) ) ;
#40400=CARTESIAN_POINT ( 'NONE',  ( 3.591611365154614877, -276.4691912798503495, -208.3696578276595233 ) ) ;
#40402=CARTESIAN_POINT ( 'NONE',  ( -53.28691492658256834, -279.7662352645559736, -340.3683826091709079 ) ) ;
#40403=CARTESIAN_POINT ( 'NONE',  ( -102.5548912273075359, -276.1799505344565659, -309.0327616309972427 ) ) ;
#40405=CARTESIAN_POINT ( 'NONE',  ( 11.95359476251294062, -281.8521149855111503, -324.2866438785825380 ) ) ;
#40406=CARTESIAN_POINT ( 'NONE',  ( -28.63086904358489804, -278.1492243804284499, -346.5204632509078806 ) ) ;
#40407=CARTESIAN_POINT ( 'NONE',  ( -15.46898969589202544, -285.3871377557672417, -196.7232530367633956 ) ) ;
#40408=CARTESIAN_POINT ( 'NONE',  ( -65.73616085099284589, -293.4357610129025602, -201.9973694044729768 ) ) ;
#40409=CARTESIAN_POINT ( 'NONE',  ( 36.11986802533294849, -277.4090978106801799, -290.6542854637510800 ) ) ;
#40410=CARTESIAN_POINT ( 'NONE',  ( 24.91578875114059244, -276.2742263817530102, -225.8718336334627566 ) ) ;
#40411=CARTESIAN_POINT ( 'NONE',  ( 13.72981172109277637, -276.1454707944167808, -322.5918520398628857 ) ) ;
#40412=CARTESIAN_POINT ( 'NONE',  ( -87.70549548037645593, -297.7577978277427633, -325.7101608088385660 ) ) ;
#40413=CARTESIAN_POINT ( 'NONE',  ( -55.16900330813625430, -283.8223120519360236, -197.6286578918427495 ) ) ;
#40414=CARTESIAN_POINT ( 'NONE',  ( 15.42676094039337009, -292.4401136461067949, -214.2412137935257306 ) ) ;
#40415=CARTESIAN_POINT ( 'NONE',  ( 16.13915119024753508, -289.9092719680049868, -324.7137803767968194 ) ) ;
#40416=CARTESIAN_POINT ( 'NONE',  ( 19.59452573732196967, -291.8217036909481976, -224.1623432967442682 ) ) ;
#40418=CARTESIAN_POINT ( 'NONE',  ( 26.01459066788044794, -291.5586767992588761, -227.5528298243347649 ) ) ;
#40419=CARTESIAN_POINT ( 'NONE',  ( -62.80412618020993420, -291.3780441841935840, -201.9231727598370298 ) ) ;
#40421=CARTESIAN_POINT ( 'NONE',  ( -20.55063799047649908, -289.9212195765249476, -345.2457274912503635 ) ) ;
#40422=CARTESIAN_POINT ( 'NONE',  ( -110.1891078100415484, -278.8099528611388678, -276.0847653329869331 ) ) ;
#40424=CARTESIAN_POINT ( 'NONE',  ( -104.3395860969774702, -294.9854890270951842, -307.7896247565028034 ) ) ;
#40425=CARTESIAN_POINT ( 'NONE',  ( -63.17500931435632339, -286.3757113337703117, -197.9321671207016493 ) ) ;
#40426=CARTESIAN_POINT ( 'NONE',  ( 18.33327024772819058, -287.1575841708763051, -217.1237175531528010 ) ) ;
#40427=CARTESIAN_POINT ( 'NONE',  ( -110.3397370399036390, -284.8421504067744650, -273.6433171318274731 ) ) ;
#40428=CARTESIAN_POINT ( 'NONE',  ( -95.79658185062278619, -239.9132554248992335, -341.7037225620111371 ) ) ;
#40429=CARTESIAN_POINT ( 'NONE',  ( 152.3546084807370846, 207.1652122862846852, -216.4903851229848613 ) ) ;
#40430=CARTESIAN_POINT ( 'NONE',  ( -77.44465942105425427, -207.6981841608007358, -353.4590041244178451 ) ) ;
#40431=CARTESIAN_POINT ( 'NONE',  ( 34.04858704456142249, -274.9606796564495426, -286.4189444767638406 ) ) ;
#40432=CARTESIAN_POINT ( 'NONE',  ( -11.15641801993444027, -275.6229932953943376, -338.8341570170778709 ) ) ;
#40433=CARTESIAN_POINT ( 'NONE',  ( -87.41745026599895141, -296.8833071322984551, -211.8790237016687570 ) ) ;
#40434=CARTESIAN_POINT ( 'NONE',  ( 139.9619883129436175, 178.0088983401332712, -238.8496011978771207 ) ) ;
#40435=CARTESIAN_POINT ( 'NONE',  ( 29.52472329102864279, -273.7507364126847165, -233.0744592506608797 ) ) ;
#40436=CARTESIAN_POINT ( 'NONE',  ( 9.890158678931786795, -300.5099204045154693, -196.1107481965832164 ) ) ;
#40438=CARTESIAN_POINT ( 'NONE',  ( -35.49103812266535130, -299.0160376997106937, -193.5961227232499198 ) ) ;
#40439=CARTESIAN_POINT ( 'NONE',  ( 35.74174720458932342, -288.0173949372725701, -268.3044774032451301 ) ) ;
#40440=CARTESIAN_POINT ( 'NONE',  ( -53.24581842444744240, -296.0537955668417567, -345.5901275544880491 ) ) ;
#40441=CARTESIAN_POINT ( 'NONE',  ( -57.37973956247277130, -298.2927415120119576, -196.0226145762185297 ) ) ;
#40442=CARTESIAN_POINT ( 'NONE',  ( -82.35814173241939784, -295.8527815415696409, -327.8931211605208773 ) ) ;
#40444=CARTESIAN_POINT ( 'NONE',  ( 28.67724042790965555, -276.9855436599220297, -233.5001720378140533 ) ) ;
#40446=CARTESIAN_POINT ( 'NONE',  ( 36.11881808418307571, -280.7722616095896910, -247.4901939255047125 ) ) ;
#40447=CARTESIAN_POINT ( 'NONE',  ( -39.15160195528284959, -278.0166744601501705, -343.5740451481016180 ) ) ;
#40448=CARTESIAN_POINT ( 'NONE',  ( 29.66027652668425318, -277.7829697282760435, -306.3151173462351835 ) ) ;
#40449=CARTESIAN_POINT ( 'NONE',  ( -97.50576853219169493, -275.9546294838840481, -315.7551121345023262 ) ) ;
#40450=CARTESIAN_POINT ( 'NONE',  ( -102.0878858124889632, -273.5060980886412949, -236.4000848177502121 ) ) ;
#40451=CARTESIAN_POINT ( 'NONE',  ( -110.3181488619163275, -295.2559180965984638, -260.4999317729956374 ) ) ;
#40453=CARTESIAN_POINT ( 'NONE',  ( -93.60467401188311953, -278.0592409012591020, -316.8939025970711896 ) ) ;
#40454=CARTESIAN_POINT ( 'NONE',  ( 7.631008024489784880, -287.1377911744011158, -332.3195218081207258 ) ) ;
#40455=CARTESIAN_POINT ( 'NONE',  ( -88.80940629332599201, -275.3300913463501729, -215.7367503887411431 ) ) ;
#40457=CARTESIAN_POINT ( 'NONE',  ( -110.5290694898110786, -289.7745044645415078, -268.4473571145647952 ) ) ;
#40458=CARTESIAN_POINT ( 'NONE',  ( -108.9305434241827868, -284.2587602294238422, -242.1387700534701253 ) ) ;
#40459=CARTESIAN_POINT ( 'NONE',  ( 14.62036482676534277, -280.5487155508267847, -323.1392121425904520 ) ) ;
#40460=CARTESIAN_POINT ( 'NONE',  ( 21.81336857316339817, -279.5178411778748568, -226.5671628940422977 ) ) ;
#40461=CARTESIAN_POINT ( 'NONE',  ( -110.6060182635314817, -282.8033965623482686, -257.1117573864958672 ) ) ;
#40462=CARTESIAN_POINT ( 'NONE',  ( -92.75689809185595891, -287.2583514653211978, -219.7476696729253831 ) ) ;
#40463=CARTESIAN_POINT ( 'NONE',  ( -108.3606650943867038, -280.0011652209780095, -251.7796529776460375 ) ) ;
#40465=CARTESIAN_POINT ( 'NONE',  ( -58.40212359098838846, -293.7800610223805506, -198.3787645216934550 ) ) ;
#40466=CARTESIAN_POINT ( 'NONE',  ( -84.25855566230353588, -275.9269049178594173, -330.2007504250416332 ) ) ;
#40468=CARTESIAN_POINT ( 'NONE',  ( 20.10771294275045307, -276.8405362612841145, -315.5858990672146547 ) ) ;
#40469=CARTESIAN_POINT ( 'NONE',  ( -109.7191243327464889, -286.2919024100184515, -290.6474901065458880 ) ) ;
#40471=CARTESIAN_POINT ( 'NONE',  ( -98.68660627855595635, -291.8761455077942060, -314.4980886571906922 ) ) ;
#40472=CARTESIAN_POINT ( 'NONE',  ( -110.3999686194082273, -294.7703480519206209, -253.3500042728492474 ) ) ;
#40473=CARTESIAN_POINT ( 'NONE',  ( 11.98177109736971424, -285.9145420156942237, -211.3734829468599798 ) ) ;
#40474=CARTESIAN_POINT ( 'NONE',  ( -72.99576474426503125, -289.9715889860896141, -205.6876940265083817 ) ) ;
#40476=CARTESIAN_POINT ( 'NONE',  ( -29.67854612603656506, -275.6380597814648468, -343.5049080530640140 ) ) ;
#40477=CARTESIAN_POINT ( 'NONE',  ( 31.72622290130566114, -292.0512403567969386, -297.7135479350594096 ) ) ;
#40480=CARTESIAN_POINT ( 'NONE',  ( -74.32575318812952503, -290.0494452150384177, -203.6161738099156651 ) ) ;
#40481=CARTESIAN_POINT ( 'NONE',  ( -97.23588749016070665, -286.7489214668028694, -227.2219598302695829 ) ) ;
#40482=CARTESIAN_POINT ( 'NONE',  ( 18.85946758155182934, -286.4965487575751695, -321.5215008779105688 ) ) ;
#40484=CARTESIAN_POINT ( 'NONE',  ( -95.43329365003492626, -286.6090191479946725, -225.1660816910496976 ) ) ;
#40486=CARTESIAN_POINT ( 'NONE',  ( -72.46048734633099286, -286.3775635797292125, -206.1653101529586252 ) ) ;
#40487=CARTESIAN_POINT ( 'NONE',  ( 28.03584519350161486, -295.0345271441481714, -232.8886832041147272 ) ) ;
#40488=CARTESIAN_POINT ( 'NONE',  ( -81.72064975485658067, -275.7311126363377412, -331.5152104494140417 ) ) ;
#40489=CARTESIAN_POINT ( 'NONE',  ( 1.040175331164154837, -276.8881083073920877, -337.1492061974268495 ) ) ;
#40490=CARTESIAN_POINT ( 'NONE',  ( 28.23820088301792808, -291.1351089485606849, -232.8299205701479480 ) ) ;
#40491=CARTESIAN_POINT ( 'NONE',  ( -113.7171041604738235, -278.6796328718843370, -260.1678642953070266 ) ) ;
#40492=CARTESIAN_POINT ( 'NONE',  ( -110.9009413954952947, -298.6956820249556017, -257.6770796488139581 ) ) ;
#40495=CARTESIAN_POINT ( 'NONE',  ( 26.80594827739740182, -285.7484557002154588, -234.3916127602344375 ) ) ;
#40496=CARTESIAN_POINT ( 'NONE',  ( -93.67924623238455695, -276.0149791513286459, -318.7030912706692334 ) ) ;
#40497=CARTESIAN_POINT ( 'NONE',  ( 7.979459066525541822, -280.4325612937215055, -330.1189055501071152 ) ) ;
#40499=CARTESIAN_POINT ( 'NONE',  ( 35.92565659406344025, -273.7601160794806106, -248.8549011955632011 ) ) ;
#40500=CARTESIAN_POINT ( 'NONE',  ( 36.40189667974279075, -295.0772904531303311, -270.7443910423835973 ) ) ;
#40501=CARTESIAN_POINT ( 'NONE',  ( 10.64036638886969399, -279.6174766508252105, -210.4665103505161881 ) ) ;
#40502=CARTESIAN_POINT ( 'NONE',  ( -0.6296499342777925889, -295.4931339881433701, -333.7880307336682790 ) ) ;
#40503=CARTESIAN_POINT ( 'NONE',  ( -43.26837292597443962, -299.2940981986686211, -194.0313000994881918 ) ) ;
#40504=CARTESIAN_POINT ( 'NONE',  ( -49.95183219354460391, -297.7200718570109075, -198.4585132051433050 ) ) ;
#40505=CARTESIAN_POINT ( 'NONE',  ( -96.71282231959645515, -293.1802604351744321, -224.5345917946154657 ) ) ;
#40506=CARTESIAN_POINT ( 'NONE',  ( -114.2082025277494495, -284.6518129132633135, -275.7198953307047873 ) ) ;
#40507=CARTESIAN_POINT ( 'NONE',  ( 31.88146062820246840, -274.0912307523720415, -301.1581875313318619 ) ) ;
#40508=CARTESIAN_POINT ( 'NONE',  ( 22.40379876867637066, -288.0373573276025354, -318.9562992615146300 ) ) ;
#40509=CARTESIAN_POINT ( 'NONE',  ( -109.5704045308657300, -280.7758564129747469, -251.4730877253806227 ) ) ;
#40511=CARTESIAN_POINT ( 'NONE',  ( 33.25927934050767476, -286.3545114275828496, -250.8955035135419394 ) ) ;
#40513=CARTESIAN_POINT ( 'NONE',  ( -70.00311722843157725, -289.6217537687813319, -202.8464344932358756 ) ) ;
#40515=CARTESIAN_POINT ( 'NONE',  ( 202.9737475146022803, 296.4636489462809550, -68.70538243550777224 ) ) ;
#40516=CARTESIAN_POINT ( 'NONE',  ( -63.84906443871414439, -288.9148660919514668, -338.4987413868928456 ) ) ;
#40518=CARTESIAN_POINT ( 'NONE',  ( -113.3646300933064310, -285.3551472233727964, -281.3820153497404704 ) ) ;
#40519=CARTESIAN_POINT ( 'NONE',  ( 38.12372545427202652, -292.7882204973093963, -284.4958596535534525 ) ) ;
#40520=CARTESIAN_POINT ( 'NONE',  ( -2.771482224829393548, -282.1015196705236576, -202.4396936741175068 ) ) ;
#40521=CARTESIAN_POINT ( 'NONE',  ( 3.544184392830691088, -281.9045571321730108, -205.6329256421611831 ) ) ;
#40522=CARTESIAN_POINT ( 'NONE',  ( -99.03217298471201957, -283.8449955845227919, -309.4850459206065239 ) ) ;
#40523=CARTESIAN_POINT ( 'NONE',  ( 33.95532903960647531, -277.2497541240009014, -246.9190415777997032 ) ) ;
#40524=CARTESIAN_POINT ( 'NONE',  ( -111.5920180545969487, -296.2966965220631437, -290.7545063182770946 ) ) ;
#40525=CARTESIAN_POINT ( 'NONE',  ( -111.2551153722055943, -288.4365953186446632, -280.8767514242893526 ) ) ;
#40527=CARTESIAN_POINT ( 'NONE',  ( -55.35637588449080937, -296.7353487853002321, -199.2473648627412786 ) ) ;
#40528=ORIENTED_EDGE ( 'NONE', *, *, #72819, .T. ) ;
#40531=CARTESIAN_POINT ( 'NONE',  ( -101.6327459194991008, -285.9672571081932233, -307.8841192875752313 ) ) ;
#40532=CARTESIAN_POINT ( 'NONE',  ( 35.19854032246905717, -294.9485850551409953, -295.4118100418284598 ) ) ;
#40533=CARTESIAN_POINT ( 'NONE',  ( -24.03881859366369866, -283.5291427728764688, -342.2424508217943639 ) ) ;
#40535=CARTESIAN_POINT ( 'NONE',  ( -14.67065778551407007, -275.8242278882383971, -343.7573731311840675 ) ) ;
#40536=CARTESIAN_POINT ( 'NONE',  ( -61.66421543717697773, -292.3957656360024657, -197.3548582175833133 ) ) ;
#40537=CARTESIAN_POINT ( 'NONE',  ( -109.7385879705670959, -282.9788843252323431, -247.8464965693437136 ) ) ;
#40538=CARTESIAN_POINT ( 'NONE',  ( 34.44157193075682954, -293.5314807704896225, -242.4126424116990961 ) ) ;
#40539=CARTESIAN_POINT ( 'NONE',  ( -110.3581415829500685, -290.8745066167260802, -271.1898302038484871 ) ) ;
#40541=CARTESIAN_POINT ( 'NONE',  ( 144.2857639756989272, -299.5541904835127980, -195.3611179825600175 ) ) ;
#40542=CARTESIAN_POINT ( 'NONE',  ( -110.7270578385798956, -271.3603141859142625, -270.3459430301334123 ) ) ;
#40543=CARTESIAN_POINT ( 'NONE',  ( -66.29508407243339718, -284.9444860100746268, -340.9755235858550577 ) ) ;
#40544=CARTESIAN_POINT ( 'NONE',  ( 10.64812456238590777, -290.1952119285920162, -210.2361428286349110 ) ) ;
#40546=CARTESIAN_POINT ( 'NONE',  ( 34.78712304438143121, -280.6455069174771211, -283.5332544925073535 ) ) ;
#40547=CARTESIAN_POINT ( 'NONE',  ( 37.88410771017887413, -275.4239870848458622, -286.7573799586867267 ) ) ;
#40548=CARTESIAN_POINT ( 'NONE',  ( -80.12332178592984633, -281.4716564351134593, -208.9627363069155308 ) ) ;
#40549=CARTESIAN_POINT ( 'NONE',  ( 186.8753510093225998, 261.0767047533620371, -152.2190506625686908 ) ) ;
#40550=CARTESIAN_POINT ( 'NONE',  ( 18.74012657635215717, -279.4145279068767422, -218.4628038820436586 ) ) ;
#40551=CARTESIAN_POINT ( 'NONE',  ( -111.2370329669978304, -282.7083774618300822, -259.8099764580837814 ) ) ;
#40552=CARTESIAN_POINT ( 'NONE',  ( -111.2437865561877146, -274.6247840391680484, -253.6641989065475684 ) ) ;
#40554=CARTESIAN_POINT ( 'NONE',  ( -108.6505628435897535, -296.8348368039759748, -286.2681774248567308 ) ) ;
#40556=CARTESIAN_POINT ( 'NONE',  ( -75.21951289112031702, -290.2210918988385515, -207.3214384937482180 ) ) ;
#40557=CARTESIAN_POINT ( 'NONE',  ( -59.62753349954910220, -277.9848474905833200, -343.9590419836419528 ) ) ;
#40558=CARTESIAN_POINT ( 'NONE',  ( 15.44679013974579718, -274.8241358229439015, -219.8659723707438616 ) ) ;
#40559=CARTESIAN_POINT ( 'NONE',  ( 36.58396856470844227, -274.7297310031748907, -290.8180893102337450 ) ) ;
#40561=CARTESIAN_POINT ( 'NONE',  ( -36.25426203478412646, -272.0655934628214254, -195.3563857614199435 ) ) ;
#40565=CARTESIAN_POINT ( 'NONE',  ( -26.68430800845607109, -283.9932177593421443, -342.9429474339771104 ) ) ;
#40566=CARTESIAN_POINT ( 'NONE',  ( 8.614004824853640940, -284.1922577934084870, -330.8759689996251723 ) ) ;
#40567=CARTESIAN_POINT ( 'NONE',  ( -109.0811241229871911, -283.7156780926910642, -284.4091681444114670 ) ) ;
#40568=CARTESIAN_POINT ( 'NONE',  ( -39.19808882758704982, -275.4757051602846900, -344.1377690184856988 ) ) ;
#40569=CARTESIAN_POINT ( 'NONE',  ( 21.16892235343681250, -284.0457944349898298, -316.0488903129968321 ) ) ;
#40570=CARTESIAN_POINT ( 'NONE',  ( -101.1931572631044105, -276.5310926147301416, -307.2563026382189832 ) ) ;
#40572=CARTESIAN_POINT ( 'NONE',  ( 20.91885401849723536, -276.0084445527244270, -225.8440116718224999 ) ) ;
#40574=CARTESIAN_POINT ( 'NONE',  ( -72.44218635038427578, -280.4024167310073494, -201.9936276683974086 ) ) ;
#40578=CARTESIAN_POINT ( 'NONE',  ( -104.3508886181872271, -286.8777724704187335, -234.8923316433779291 ) ) ;
#40579=CARTESIAN_POINT ( 'NONE',  ( -72.21052236660966628, -294.7230507547126308, -334.6931227954037240 ) ) ;
#40580=CARTESIAN_POINT ( 'NONE',  ( -96.31822571377115594, -289.2355750275310129, -319.7280971465426660 ) ) ;
#40581=CARTESIAN_POINT ( 'NONE',  ( 36.66826209343179244, -285.8011989209114745, -271.0678731423714680 ) ) ;
#40582=CARTESIAN_POINT ( 'NONE',  ( -44.06024607761280976, -284.5402646378329337, -197.0792235106676173 ) ) ;
#40583=CARTESIAN_POINT ( 'NONE',  ( -60.55582111289538005, -289.9868797404074030, -200.0287696616872779 ) ) ;
#40585=CARTESIAN_POINT ( 'NONE',  ( -100.7364163632577743, -285.2522939534815123, -307.3508524710385359 ) ) ;
#40586=CARTESIAN_POINT ( 'NONE',  ( 36.75576178132580907, -273.4019796768719175, -258.6778656054111138 ) ) ;
#40587=CARTESIAN_POINT ( 'NONE',  ( 38.55977574400233010, -285.8596861223417136, -263.0544528729133731 ) ) ;
#40588=CARTESIAN_POINT ( 'NONE',  ( -72.36982823571389645, -299.5891824997087838, -203.9861367232120983 ) ) ;
#40589=CARTESIAN_POINT ( 'NONE',  ( 20.07181748108543573, -286.2215906927706897, -318.8762334154830000 ) ) ;
#40590=CARTESIAN_POINT ( 'NONE',  ( 20.69506519269020117, -281.8665436756331815, -225.6737248417511807 ) ) ;
#40591=CARTESIAN_POINT ( 'NONE',  ( -88.23111489452762157, -291.7630158040153674, -325.6810591336947596 ) ) ;
#40594=CARTESIAN_POINT ( 'NONE',  ( -71.40261072835853895, -297.4185974406583455, -337.8086425525673917 ) ) ;
#40595=CARTESIAN_POINT ( 'NONE',  ( -99.64110039250881812, -277.1176352738476680, -228.5102880108437660 ) ) ;
#40596=CARTESIAN_POINT ( 'NONE',  ( 20.26442346843702680, -292.0591352435089902, -219.4915230163975082 ) ) ;
#40597=CARTESIAN_POINT ( 'NONE',  ( -77.93519425016025082, -295.8969572855212391, -208.6668662079475780 ) ) ;
#40598=CARTESIAN_POINT ( 'NONE',  ( 12.23711621012914996, -281.0294206572767735, -324.6122419106225152 ) ) ;
#40599=CARTESIAN_POINT ( 'NONE',  ( 14.51702123860494531, -272.8686128865963951, -216.9571179955988214 ) ) ;
#40600=CARTESIAN_POINT ( 'NONE',  ( 29.17779792781686510, -294.4466323721616163, -238.9936709406285331 ) ) ;
#40601=CARTESIAN_POINT ( 'NONE',  ( -54.49178911615188525, -294.3376638359845288, -195.3683826091709363 ) ) ;
#40602=CARTESIAN_POINT ( 'NONE',  ( -109.6945093321504459, -294.7239762540878587, -294.6052668116122391 ) ) ;
#40603=CARTESIAN_POINT ( 'NONE',  ( 37.33360845913221482, -291.6138812920016221, -256.3050764695099133 ) ) ;
#40604=CARTESIAN_POINT ( 'NONE',  ( -99.32839922685357692, -291.4331961887654074, -310.0224852261586648 ) ) ;
#40606=CARTESIAN_POINT ( 'NONE',  ( -17.39837761794011683, -293.1188738049671088, -199.9176053912980819 ) ) ;
#40607=CARTESIAN_POINT ( 'NONE',  ( -2.419275701860534422, -280.6125310240805106, -337.1355972223573758 ) ) ;
#40608=CARTESIAN_POINT ( 'NONE',  ( -36.20613000907598433, -292.0667459473677354, -197.3574743847684942 ) ) ;
#40609=CARTESIAN_POINT ( 'NONE',  ( 35.32768634397170615, -281.2292449773694898, -244.7428761329562690 ) ) ;
#40610=CARTESIAN_POINT ( 'NONE',  ( -95.32160518925131498, -283.5338528613874587, -320.9978131815226448 ) ) ;
#40611=CARTESIAN_POINT ( 'NONE',  ( -15.33625967234313592, -286.7665914083011671, -341.9400072225873828 ) ) ;
#40612=CARTESIAN_POINT ( 'NONE',  ( -15.79625802500858534, -280.9100225573880607, -341.4009617520089819 ) ) ;
#40613=CARTESIAN_POINT ( 'NONE',  ( -38.14302996174868099, -278.5221656627724087, -194.0586565157570078 ) ) ;
#40614=CARTESIAN_POINT ( 'NONE',  ( 3.005770047155969404, -287.4446158750764084, -335.6428392101049099 ) ) ;
#40616=CARTESIAN_POINT ( 'NONE',  ( 20.80070679906746989, -294.5182937766302871, -224.8884830366427252 ) ) ;
#40617=CARTESIAN_POINT ( 'NONE',  ( -35.70578721796089638, -278.4573057941085494, -346.7674003240754246 ) ) ;
#40618=CARTESIAN_POINT ( 'NONE',  ( -37.81415524445844767, -276.7249124765496617, -343.3931900727663447 ) ) ;
#40619=CARTESIAN_POINT ( 'NONE',  ( 39.50230333779012426, -293.7898169480481556, -276.0370319631380198 ) ) ;
#40620=CARTESIAN_POINT ( 'NONE',  ( -76.04178007673230866, -281.6443055688143886, -335.3187718231940266 ) ) ;
#40621=CARTESIAN_POINT ( 'NONE',  ( 34.00192346484114836, -292.8290136197932156, -286.9540339595770888 ) ) ;
#40623=CARTESIAN_POINT ( 'NONE',  ( -111.4102552849610959, -294.7043319699102994, -258.4964773301505829 ) ) ;
#40626=CARTESIAN_POINT ( 'NONE',  ( 35.68303615358379943, -293.0292401754815614, -268.0424260105511962 ) ) ;
#40627=CARTESIAN_POINT ( 'NONE',  ( -102.0172624299487154, -282.4809262143061233, -239.1787733560258289 ) ) ;
#40628=CARTESIAN_POINT ( 'NONE',  ( -57.31690184651372988, -296.8593730560855306, -196.1857602132345733 ) ) ;
#40629=CARTESIAN_POINT ( 'NONE',  ( 37.04651610637017001, -279.5090048715456987, -255.9840957467037299 ) ) ;
#40630=CARTESIAN_POINT ( 'NONE',  ( 4.893391828027300328, -287.9246822947409328, -206.5054303329810637 ) ) ;
#40631=CARTESIAN_POINT ( 'NONE',  ( -82.54792958280471282, -289.5231336466910079, -327.6794991789068945 ) ) ;
#40632=CARTESIAN_POINT ( 'NONE',  ( -110.6579623673950294, -280.1759807848645778, -262.4254115385907085 ) ) ;
#40633=CARTESIAN_POINT ( 'NONE',  ( -76.54284540983506702, -293.5990747032025183, -333.9439604949582758 ) ) ;
#40634=CARTESIAN_POINT ( 'NONE',  ( 53.20184915273028281, -300.9609013388575249, -196.3202096819806002 ) ) ;
#40635=CARTESIAN_POINT ( 'NONE',  ( -108.8767090927624679, -277.1308054369759475, -286.8446781887727184 ) ) ;
#40637=CARTESIAN_POINT ( 'NONE',  ( -31.90712548919840685, -297.7851723854034276, -193.3825591744275982 ) ) ;
#40638=CARTESIAN_POINT ( 'NONE',  ( -107.0678953280349219, -292.8150604373320220, -244.1461216927069700 ) ) ;
#40639=CARTESIAN_POINT ( 'NONE',  ( 21.68005793977844320, -295.8061720122201450, -318.5777965286123958 ) ) ;
#40641=CARTESIAN_POINT ( 'NONE',  ( -109.5184244067401664, -291.0498052471228903, -282.0334650613423264 ) ) ;
#40644=CARTESIAN_POINT ( 'NONE',  ( -89.54520047544303907, -297.9910159113310897, -213.8256508201602344 ) ) ;
#40645=CARTESIAN_POINT ( 'NONE',  ( -100.6387728551556080, -289.2491460361017630, -228.6282578355832129 ) ) ;
#40647=CARTESIAN_POINT ( 'NONE',  ( -100.7356617306175082, -297.4623617054941178, -226.6693137411275529 ) ) ;
#40650=CARTESIAN_POINT ( 'NONE',  ( 0.3934302980274854145, -290.0794218272779403, -336.7440416135048622 ) ) ;
#40651=CARTESIAN_POINT ( 'NONE',  ( -2.602324593224680793, -285.1233781216987495, -342.4248175857292154 ) ) ;
#40652=CARTESIAN_POINT ( 'NONE',  ( -111.8216786182747029, -286.6523929862374871, -262.5842240417235871 ) ) ;
#40653=CARTESIAN_POINT ( 'NONE',  ( 38.39367995880343187, -285.9991284681446473, -260.2241314648887283 ) ) ;
#40654=CARTESIAN_POINT ( 'NONE',  ( -27.01254004751618609, -272.1834772602756516, -196.1918913530755333 ) ) ;
#40655=CARTESIAN_POINT ( 'NONE',  ( -105.7117979925263143, -274.8618111726309508, -240.7881760963864792 ) ) ;
#40656=CARTESIAN_POINT ( 'NONE',  ( -104.8521996805456382, -289.0471803197867757, -238.9979764772720330 ) ) ;
#40657=CARTESIAN_POINT ( 'NONE',  ( -97.80316935413354429, -279.7943165631121474, -316.0410954951530584 ) ) ;
#40659=CARTESIAN_POINT ( 'NONE',  ( -54.49278902472478592, -279.8257284137872034, -199.3523133290802889 ) ) ;
#40660=CARTESIAN_POINT ( 'NONE',  ( 30.11874429890719185, -280.5235231508592619, -242.2011977837823622 ) ) ;
#40661=CARTESIAN_POINT ( 'NONE',  ( 30.27703999937892121, -277.1026094226147052, -306.6561325203267643 ) ) ;
#40662=CARTESIAN_POINT ( 'NONE',  ( -1.308577264840212084, -279.3142500762873510, -202.7621329596578619 ) ) ;
#40663=CARTESIAN_POINT ( 'NONE',  ( 200.9738562182569694, 293.9636489450776367, -53.99999999999825917 ) ) ;
#40664=CARTESIAN_POINT ( 'NONE',  ( 33.97014131456837305, -276.8566111095771589, -298.9200024418319117 ) ) ;
#40667=CARTESIAN_POINT ( 'NONE',  ( -1.643150907947507955, -276.0366957834737036, -202.9198743873436115 ) ) ;
#40668=CARTESIAN_POINT ( 'NONE',  ( -54.49178911615187815, -294.3376638359846424, -195.3683826091709363 ) ) ;
#40669=EDGE_LOOP ( 'NONE', ( #62976, #23068, #88765, #8866 ) ) ;
#40671=CARTESIAN_POINT ( 'NONE',  ( -3.210252635886408079, -289.6702356716222653, -335.2962361339669428 ) ) ;
#40672=CARTESIAN_POINT ( 'NONE',  ( 36.84063434880250298, -289.5216498450827771, -286.8813165054038450 ) ) ;
#40673=CARTESIAN_POINT ( 'NONE',  ( -95.03612878912406359, -289.2689279304526622, -315.2728316886317543 ) ) ;
#40674=CARTESIAN_POINT ( 'NONE',  ( -67.15941828578772288, -285.1792073163438204, -199.4355895234700142 ) ) ;
#40676=CARTESIAN_POINT ( 'NONE',  ( 33.72437283331294822, -280.2122097568085337, -290.2622156956471144 ) ) ;
#40677=CARTESIAN_POINT ( 'NONE',  ( 20.49042084099458805, -290.0596203061363667, -316.9047670461927737 ) ) ;
#40678=CARTESIAN_POINT ( 'NONE',  ( 10.34273089995996919, -280.8603152822681182, -326.6145316231485936 ) ) ;
#40679=CARTESIAN_POINT ( 'NONE',  ( -77.10264685039649635, -280.8225987254154461, -208.4917825281967794 ) ) ;
#40680=CARTESIAN_POINT ( 'NONE',  ( -66.82174787274989569, -277.9415405047414538, -337.2110635830526348 ) ) ;
#40681=CARTESIAN_POINT ( 'NONE',  ( -113.7178966205537449, -289.2648225317471429, -276.9043214449955030 ) ) ;
#40682=CARTESIAN_POINT ( 'NONE',  ( -112.3652097174486073, -285.1469110143468697, -286.9632814028813641 ) ) ;
#40683=CARTESIAN_POINT ( 'NONE',  ( -67.85118003366478945, -283.9343592434242964, -340.9918374979868076 ) ) ;
#40684=CARTESIAN_POINT ( 'NONE',  ( 29.31532614387689151, -282.1211010912938377, -300.2483198753235456 ) ) ;
#40687=CARTESIAN_POINT ( 'NONE',  ( -110.0535167177606155, -292.6839593943728346, -249.0703404102804654 ) ) ;
#40688=CARTESIAN_POINT ( 'NONE',  ( 24.42627313287446000, -291.6337850748248570, -225.2167301482050163 ) ) ;
#40689=CARTESIAN_POINT ( 'NONE',  ( -0.4173147049840161826, -273.6147202248304211, -207.1009397883750296 ) ) ;
#40690=CARTESIAN_POINT ( 'NONE',  ( -33.44830585809430801, -294.3529690140140929, -347.1736618969711685 ) ) ;
#40691=CARTESIAN_POINT ( 'NONE',  ( -93.96021457574521207, -289.6952014970873392, -223.1709725755519855 ) ) ;
#40692=CARTESIAN_POINT ( 'NONE',  ( -10.13811898126777145, -292.9319344913764667, -339.1938077947906436 ) ) ;
#40693=CARTESIAN_POINT ( 'NONE',  ( -37.25221129623628258, -290.2560850006350393, -343.7581376632795696 ) ) ;
#40694=DIRECTION ( 'NONE',  ( -1.000000000000000000, -0.000000000000000000, -0.000000000000000000 ) ) ;
#40695=CARTESIAN_POINT ( 'NONE',  ( -98.23125718123426964, -291.9561389976308874, -314.1719512147217301 ) ) ;
#40696=CARTESIAN_POINT ( 'NONE',  ( -6.612550951882577799, -290.4544925747460979, -201.7487136718380611 ) ) ;
#40697=CARTESIAN_POINT ( 'NONE',  ( 35.89474624726534557, -295.7605949643664189, -286.5878766716460859 ) ) ;
#40698=CARTESIAN_POINT ( 'NONE',  ( -94.31261987028145199, -286.1423031798886996, -224.3225163270527958 ) ) ;
#40699=CARTESIAN_POINT ( 'NONE',  ( 24.22794957966838680, -296.1366013379931132, -313.5021101504153194 ) ) ;
#40700=CARTESIAN_POINT ( 'NONE',  ( -46.70221885926734728, -275.9137635942802262, -195.5895492525627049 ) ) ;
#40701=CARTESIAN_POINT ( 'NONE',  ( 20.51024390910566098, -275.0293340262962829, -320.5921328273016115 ) ) ;
#40702=CARTESIAN_POINT ( 'NONE',  ( -35.82182847936549308, -297.2678989818052742, -193.5227940414692682 ) ) ;
#40703=CARTESIAN_POINT ( 'NONE',  ( -54.20631320576049461, -275.5114118493416981, -342.4803362891933034 ) ) ;
#40704=CARTESIAN_POINT ( 'NONE',  ( -72.79440827390649815, -277.6585137550201807, -204.9056393367679902 ) ) ;
#40705=CARTESIAN_POINT ( 'NONE',  ( -81.32113580075613868, -274.6444572359360450, -211.5356136496031922 ) ) ;
#40706=CARTESIAN_POINT ( 'NONE',  ( -18.67620321177383502, -272.8625595547588887, -196.2105848871857461 ) ) ;
#40707=CARTESIAN_POINT ( 'NONE',  ( -109.6278670026663491, -298.1587260822187773, -256.5067882255931409 ) ) ;
#40709=CARTESIAN_POINT ( 'NONE',  ( -69.33736392543778493, -298.4228197239996234, -204.5668991960239964 ) ) ;
#40712=CARTESIAN_POINT ( 'NONE',  ( -71.19072634182349191, -287.5168853751376332, -337.6860779236608323 ) ) ;
#40713=CARTESIAN_POINT ( 'NONE',  ( -100.7167115039422214, -272.8831171082964602, -234.0295411440080500 ) ) ;
#40714=CARTESIAN_POINT ( 'NONE',  ( 20.28674988660977263, -286.8596702667462068, -219.2142027799276889 ) ) ;
#40716=CARTESIAN_POINT ( 'NONE',  ( -26.15182502095681727, -288.5801221705755779, -346.5223350588607900 ) ) ;
#40717=CARTESIAN_POINT ( 'NONE',  ( -112.3043731446424545, -298.4338816474951841, -278.0425537548256330 ) ) ;
#40718=CARTESIAN_POINT ( 'NONE',  ( -34.25032877576914103, -293.0130252935406361, -345.1305759983741837 ) ) ;
#40720=CARTESIAN_POINT ( 'NONE',  ( 19.65684331992298794, -281.4512309075841472, -321.9687939641002572 ) ) ;
#40723=CARTESIAN_POINT ( 'NONE',  ( -112.3830721958973413, -276.5362639220081746, -271.5856794472763909 ) ) ;
#40725=CARTESIAN_POINT ( 'NONE',  ( -48.13445022982620713, -287.9873033114513419, -343.0116405947665612 ) ) ;
#40727=CARTESIAN_POINT ( 'NONE',  ( -95.67549732217206326, -287.9030632420486882, -317.5010029872674409 ) ) ;
#40728=CARTESIAN_POINT ( 'NONE',  ( -80.20910950928154648, -299.0608441273629978, -210.2876161177727568 ) ) ;
#40729=CARTESIAN_POINT ( 'NONE',  ( 34.76556382236587694, -282.6542875849948473, -244.9218044263096488 ) ) ;
#40730=CARTESIAN_POINT ( 'NONE',  ( -43.13754190542001510, -295.9995636395456131, -195.1770607610970103 ) ) ;
#40731=CARTESIAN_POINT ( 'NONE',  ( -95.92174313203582869, -283.9411625859445962, -313.9200270788040257 ) ) ;
#40732=CARTESIAN_POINT ( 'NONE',  ( -31.30935756776330336, -275.5550739934492412, -197.0067972287041869 ) ) ;
#40733=CARTESIAN_POINT ( 'NONE',  ( 36.02281967335061807, -283.3515133523521285, -254.7226156802384480 ) ) ;
#40734=CARTESIAN_POINT ( 'NONE',  ( -60.57923519024238601, -296.8020830102483956, -200.8565948379476822 ) ) ;
#40736=CARTESIAN_POINT ( 'NONE',  ( 204.8722290845309431, 293.3206796832986925, -54.00000000000338929 ) ) ;
#40737=CARTESIAN_POINT ( 'NONE',  ( -8.390006710344874108, -294.5169032120475094, -341.7674372384428807 ) ) ;
#40738=CARTESIAN_POINT ( 'NONE',  ( -96.27075699170869427, -287.1635492943576082, -224.5231848368011924 ) ) ;
#40740=CARTESIAN_POINT ( 'NONE',  ( -115.3288506153726871, -282.2666405000203440, -252.5284128619063608 ) ) ;
#40741=CARTESIAN_POINT ( 'NONE',  ( -108.5107275564088098, -277.3806568782591171, -299.3288302666456957 ) ) ;
#40742=CARTESIAN_POINT ( 'NONE',  ( -107.0083240628469525, -288.5524772779304499, -301.3617035926965855 ) ) ;
#40743=CARTESIAN_POINT ( 'NONE',  ( -103.6279268527864588, -285.6390550488317217, -302.6783089496187813 ) ) ;
#40744=CARTESIAN_POINT ( 'NONE',  ( -59.47699923191905214, -279.1028905083606446, -340.9869103347682540 ) ) ;
#40745=CARTESIAN_POINT ( 'NONE',  ( -113.7516335173012436, -285.9819387223919875, -270.0028293630546727 ) ) ;
#40746=CARTESIAN_POINT ( 'NONE',  ( -34.84834122616985042, -281.8150925183938966, -343.7283336771308200 ) ) ;
#40747=CARTESIAN_POINT ( 'NONE',  ( -46.73143214481503804, -281.9332393483321084, -195.8987116322781503 ) ) ;
#40748=CARTESIAN_POINT ( 'NONE',  ( -31.26218179661070806, -274.2935900508747977, -193.5882153225365698 ) ) ;
#40749=CARTESIAN_POINT ( 'NONE',  ( -25.77206355675157923, -276.7419733318878912, -346.4869579719969011 ) ) ;
#40750=CARTESIAN_POINT ( 'NONE',  ( -97.55916704965966346, -297.8714093582178748, -314.1455308458188824 ) ) ;
#40753=CARTESIAN_POINT ( 'NONE',  ( -110.4072122214023040, -294.4365812169259584, -290.4044815935360475 ) ) ;
#40754=CARTESIAN_POINT ( 'NONE',  ( 34.76685974822430580, -275.2188592174068731, -282.4286251204140399 ) ) ;
#40755=CARTESIAN_POINT ( 'NONE',  ( -82.79846264992411875, -298.5267956779829319, -208.5280224608817150 ) ) ;
#40756=CARTESIAN_POINT ( 'NONE',  ( -1.718066948587068987, -288.2907742959700386, -205.4273493023209767 ) ) ;
#40757=CARTESIAN_POINT ( 'NONE',  ( 30.29679852815585406, -295.5321171716436197, -305.6844990564229647 ) ) ;
#40758=CARTESIAN_POINT ( 'NONE',  ( 38.84386646662502329, -294.8637600141316284, -278.8356150261316202 ) ) ;
#40759=CARTESIAN_POINT ( 'NONE',  ( -107.4366345674533676, -292.8950539676741300, -244.0084363771255767 ) ) ;
#40760=CARTESIAN_POINT ( 'NONE',  ( -69.28327963476367302, -277.6307593934475904, -202.6871648721881058 ) ) ;
#40761=CARTESIAN_POINT ( 'NONE',  ( -94.20572702861829839, -281.1419522914044364, -222.3019699944966021 ) ) ;
#40762=CARTESIAN_POINT ( 'NONE',  ( -97.58796398658721216, -294.0317217691893461, -314.1058973431291861 ) ) ;
#40763=CARTESIAN_POINT ( 'NONE',  ( -97.05603242901973715, -285.7792979252941450, -316.9926952909643205 ) ) ;
#40764=CARTESIAN_POINT ( 'NONE',  ( -14.45651033147271391, -285.2761118086507395, -200.6623818813432081 ) ) ;
#40765=CARTESIAN_POINT ( 'NONE',  ( 155.5252760472149873, 205.5130994547002388, -216.6222576925314343 ) ) ;
#40766=EDGE_LOOP ( 'NONE', ( #48982, #2246, #36979, #28598 ) ) ;
#40767=CARTESIAN_POINT ( 'NONE',  ( -98.12231486432158079, -284.7805100993483052, -229.8913223435700672 ) ) ;
#40769=CARTESIAN_POINT ( 'NONE',  ( 28.04866328337839576, -283.1585939237264711, -310.5316349792955180 ) ) ;
#40770=CARTESIAN_POINT ( 'NONE',  ( -71.92148776104070862, -273.9153231682902856, -205.9905027090790668 ) ) ;
#40771=CARTESIAN_POINT ( 'NONE',  ( 24.39242218744337976, -285.7415533311229296, -225.0079829049096816 ) ) ;
#40772=CARTESIAN_POINT ( 'NONE',  ( -39.59240733921521382, -280.9658174499913912, -193.6164024688690972 ) ) ;
#40773=DIRECTION ( 'NONE',  ( 0.000000000000000000, 0.000000000000000000, 1.000000000000000000 ) ) ;
#40774=CARTESIAN_POINT ( 'NONE',  ( -79.54359671755467787, -281.0137518218346031, -206.7232973948598556 ) ) ;
#40775=CARTESIAN_POINT ( 'NONE',  ( 20.04707733962005278, -281.5085053594997930, -219.1569386987120538 ) ) ;
#40776=CARTESIAN_POINT ( 'NONE',  ( 17.40634833298269157, -284.4094976428775112, -226.7417163044926838 ) ) ;
#40778=CARTESIAN_POINT ( 'NONE',  ( -70.32131025625263021, -275.6166088378918744, -203.1869135081190620 ) ) ;
#40779=CARTESIAN_POINT ( 'NONE',  ( -114.2130631985986611, -273.1142508670334337, -284.1207669014788166 ) ) ;
#40780=AXIS2_PLACEMENT_3D ( 'NONE', #65321, #13710, #6610 ) ;
#40781=CARTESIAN_POINT ( 'NONE',  ( -27.31297884136561294, -278.2001842557492068, -196.3407276125316230 ) ) ;
#40782=CARTESIAN_POINT ( 'NONE',  ( 37.32528725606848496, -295.1335947456945519, -256.2609403032764703 ) ) ;
#40783=CARTESIAN_POINT ( 'NONE',  ( -72.18045306765381497, -294.8744456583661986, -334.6416815503314979 ) ) ;
#40784=CARTESIAN_POINT ( 'NONE',  ( -97.41158513264095120, -290.7042885283434543, -222.2868439980655921 ) ) ;
#40785=CARTESIAN_POINT ( 'NONE',  ( 115.2448031289451222, -299.5541904835127980, -195.3611179825600175 ) ) ;
#40786=CARTESIAN_POINT ( 'NONE',  ( -79.16970383640156683, -294.1794160040460611, -334.3065978670253457 ) ) ;
#40787=CARTESIAN_POINT ( 'NONE',  ( 35.74988827704921590, -286.0863260417717129, -280.6539328188176228 ) ) ;
#40788=CARTESIAN_POINT ( 'NONE',  ( 21.96659234642915237, -294.7959920027644216, -225.7137000664298796 ) ) ;
#40789=CARTESIAN_POINT ( 'NONE',  ( 35.94225504082317713, -286.3179257838690432, -276.5393517682699098 ) ) ;
#40790=CARTESIAN_POINT ( 'NONE',  ( -110.4869636751025865, -285.9675168945678365, -262.7152819765586287 ) ) ;
#40792=CARTESIAN_POINT ( 'NONE',  ( -30.72952027957549959, -293.0749191594383660, -193.8291165596032783 ) ) ;
#40793=CARTESIAN_POINT ( 'NONE',  ( -42.93137296007004267, -283.6168105322291240, -343.2586489960274889 ) ) ;
#40794=CARTESIAN_POINT ( 'NONE',  ( -113.9120860140077696, -295.3926165118751328, -266.7386726728709050 ) ) ;
#40795=CARTESIAN_POINT ( 'NONE',  ( -80.44156562110758557, -290.4225811138954896, -334.0379702815916971 ) ) ;
#40796=CARTESIAN_POINT ( 'NONE',  ( -16.64919588928149352, -292.8048955457495595, -196.2574934328994516 ) ) ;
#40797=CARTESIAN_POINT ( 'NONE',  ( 32.27295258127616506, -287.4270622252837484, -248.3465597118683377 ) ) ;
#40800=CARTESIAN_POINT ( 'NONE',  ( -102.0481672979126273, -297.8894987306101143, -309.7740420733584301 ) ) ;
#40801=CARTESIAN_POINT ( 'NONE',  ( -75.51919720547898862, -296.2392189133624925, -203.9996681549014284 ) ) ;
#40802=CARTESIAN_POINT ( 'NONE',  ( 32.20381646552353061, -280.3052812333497172, -247.2484346923745591 ) ) ;
#40804=CARTESIAN_POINT ( 'NONE',  ( 34.66636598366659427, -274.7166918549107777, -243.2619423870185926 ) ) ;
#40805=CARTESIAN_POINT ( 'NONE',  ( -110.7919826542591863, -294.9460210298589118, -276.9424819505929349 ) ) ;
#40806=CARTESIAN_POINT ( 'NONE',  ( -36.42758969182520445, -278.9010281178919968, -344.6033714018661271 ) ) ;
#40807=CARTESIAN_POINT ( 'NONE',  ( -31.21453646993573727, -272.2699158702042155, -196.3663419807342336 ) ) ;
#40808=CARTESIAN_POINT ( 'NONE',  ( -72.30025978504744444, -296.7306346518647047, -334.9125038239262722 ) ) ;
#40809=CARTESIAN_POINT ( 'NONE',  ( -109.3518920008327626, -297.8131810571256324, -256.5552608076564525 ) ) ;
#40811=CARTESIAN_POINT ( 'NONE',  ( -113.1452920391883197, -298.0541790381083160, -278.1235832924380702 ) ) ;
#40812=CARTESIAN_POINT ( 'NONE',  ( -43.12272060284060871, -295.9792986173570739, -195.3651410756511666 ) ) ;
#40813=CARTESIAN_POINT ( 'NONE',  ( -67.85128520249233475, -292.2922183153227138, -203.9165132173930886 ) ) ;
#40814=CARTESIAN_POINT ( 'NONE',  ( -100.8213516803394896, -288.6186554914600606, -307.6866326828009051 ) ) ;
#40816=CARTESIAN_POINT ( 'NONE',  ( -27.01099509605257509, -274.6723510927560596, -194.0659876162978321 ) ) ;
#40817=CARTESIAN_POINT ( 'NONE',  ( -91.86350586436429921, -297.5798225096255578, -221.7868430412704015 ) ) ;
#40818=CARTESIAN_POINT ( 'NONE',  ( -20.15636797866193675, -282.2516531660892269, -196.9381063469822948 ) ) ;
#40819=CARTESIAN_POINT ( 'NONE',  ( -34.51407401549179355, -281.7021378490764505, -346.8156979919957053 ) ) ;
#40820=CARTESIAN_POINT ( 'NONE',  ( -80.17629944680187748, -276.9638439778925090, -334.2884352067326859 ) ) ;
#40821=CARTESIAN_POINT ( 'NONE',  ( -29.43734602465698558, -282.1467764117663819, -343.1449642762883059 ) ) ;
#40822=CARTESIAN_POINT ( 'NONE',  ( 24.40931763100144281, -280.1322721915568081, -313.2421186560339379 ) ) ;
#40823=CARTESIAN_POINT ( 'NONE',  ( -94.22234407881526863, -271.7832063693932128, -223.6513004685467934 ) ) ;
#40824=CARTESIAN_POINT ( 'NONE',  ( -103.3349993597024081, -280.0779075713660404, -306.1041723858960495 ) ) ;
#40827=CARTESIAN_POINT ( 'NONE',  ( -57.10427690919379273, -296.0406156110562392, -196.9348153049176631 ) ) ;
#40828=CARTESIAN_POINT ( 'NONE',  ( -39.87502861699211110, -279.0840375963972519, -345.4978420900201286 ) ) ;
#40829=CARTESIAN_POINT ( 'NONE',  ( 27.00448396442096310, -273.0349971886321896, -231.7303622426582024 ) ) ;
#40832=CARTESIAN_POINT ( 'NONE',  ( -110.0981731642692978, -286.2119089200976987, -290.7525336038329442 ) ) ;
#40835=CARTESIAN_POINT ( 'NONE',  ( 29.40140730054798723, -286.0057912162362186, -304.6840805177163247 ) ) ;
#40837=CARTESIAN_POINT ( 'NONE',  ( 14.58641805611695474, -293.0964505981641537, -322.3035668874909447 ) ) ;
#40838=CARTESIAN_POINT ( 'NONE',  ( 36.22344169838126504, -285.5577553103556738, -260.0331182147264144 ) ) ;
#40839=CARTESIAN_POINT ( 'NONE',  ( -114.4693268140674434, -273.6886850827510216, -284.2063049943780015 ) ) ;
#40840=CARTESIAN_POINT ( 'NONE',  ( -91.87860149268118448, -293.8295572229975505, -321.9211512346975610 ) ) ;
#40841=CARTESIAN_POINT ( 'NONE',  ( -100.4124057866275876, -283.6046788040872570, -227.3167484595732617 ) ) ;
#40842=CARTESIAN_POINT ( 'NONE',  ( 24.34008617122410101, -282.5954890819425600, -229.7498932956006001 ) ) ;
#40843=CARTESIAN_POINT ( 'NONE',  ( 39.30540471429771543, -288.7719187111901533, -271.5298351959435763 ) ) ;
#40844=CARTESIAN_POINT ( 'NONE',  ( 7.960616284745397842, -278.9011784544928219, -209.2901720496602991 ) ) ;
#40845=CARTESIAN_POINT ( 'NONE',  ( -84.68502914533901560, -289.7257183005926322, -325.9940982908404976 ) ) ;
#40846=CARTESIAN_POINT ( 'NONE',  ( -32.94580629236323688, -281.5338940558859804, -196.9032999153979802 ) ) ;
#40847=CARTESIAN_POINT ( 'NONE',  ( -30.25690234391162292, -280.9467639918202053, -197.4930206804950501 ) ) ;
#40848=CARTESIAN_POINT ( 'NONE',  ( 36.22481430127140101, -289.7413652231179526, -286.7411050212907071 ) ) ;
#40850=EDGE_LOOP ( 'NONE', ( #90964, #79228, #20707, #15453 ) ) ;
#40851=CARTESIAN_POINT ( 'NONE',  ( -114.1810291951405389, -272.6238746950663199, -264.6262428901742965 ) ) ;
#40853=CARTESIAN_POINT ( 'NONE',  ( -101.1299814222145983, -293.0541704589147116, -231.5938383425343545 ) ) ;
#40855=CARTESIAN_POINT ( 'NONE',  ( -55.63300648810263738, -300.3376638359844719, -190.3683826091709363 ) ) ;
#40857=CARTESIAN_POINT ( 'NONE',  ( 33.99823975984501345, -273.2447717856712757, -246.5190087516483857 ) ) ;
#40859=CARTESIAN_POINT ( 'NONE',  ( -97.65388681535674209, -294.3239000025851624, -316.9323597000637278 ) ) ;
#40860=CARTESIAN_POINT ( 'NONE',  ( -101.2653793693434920, -296.5429530137053007, -234.9810151879597129 ) ) ;
#40861=CARTESIAN_POINT ( 'NONE',  ( -26.35256064096607531, -290.4300345296048249, -343.2820336454902872 ) ) ;
#40862=CARTESIAN_POINT ( 'NONE',  ( -18.45572455530352940, -284.5657957651918082, -341.9774706403745199 ) ) ;
#40863=CARTESIAN_POINT ( 'NONE',  ( -101.7944090981691119, -291.4341600051653813, -311.5005594390137844 ) ) ;
#40864=CARTESIAN_POINT ( 'NONE',  ( -62.58503126303945407, -290.6889382953436325, -342.6395187608372339 ) ) ;
#40865=CARTESIAN_POINT ( 'NONE',  ( -7.481455919679338429, -288.4438165826724116, -201.5616523811309264 ) ) ;
#40866=CARTESIAN_POINT ( 'NONE',  ( -100.2502106458468347, -279.3063546934228611, -225.9593239990914242 ) ) ;
#40867=CARTESIAN_POINT ( 'NONE',  ( -108.0978744198313137, -294.2885667870677935, -297.0207124331947171 ) ) ;
#40868=CARTESIAN_POINT ( 'NONE',  ( -50.09559852093136101, -283.0437884431527777, -346.3514014124780260 ) ) ;
#40869=CARTESIAN_POINT ( 'NONE',  ( 36.24179311842240025, -277.2852502986532954, -260.5460784150674272 ) ) ;
#40870=CARTESIAN_POINT ( 'NONE',  ( 99.44099354567467230, -302.2645883696979467, -195.3030568020281521 ) ) ;
#40871=CARTESIAN_POINT ( 'NONE',  ( 5.284070706827503017, -274.7238545970356540, -333.2659482633400785 ) ) ;
#40873=CARTESIAN_POINT ( 'NONE',  ( -6.737924298192999650, -279.9727170801672855, -204.0044325830203320 ) ) ;
#40874=CARTESIAN_POINT ( 'NONE',  ( -93.03470374325408443, -279.0346222545300634, -323.0328254285655589 ) ) ;
#40875=CARTESIAN_POINT ( 'NONE',  ( -26.64200715918355655, -285.2437042387158499, -194.2924098185255275 ) ) ;
#40876=CARTESIAN_POINT ( 'NONE',  ( -1.974665632540484772, -294.2873757498284704, -205.3302152267432632 ) ) ;
#40877=CARTESIAN_POINT ( 'NONE',  ( 21.22280191546856898, -276.4896502891693899, -221.6103280585869015 ) ) ;
#40878=CARTESIAN_POINT ( 'NONE',  ( -32.72917726941999206, -275.4242773834973264, -193.9803691665565566 ) ) ;
#40880=CARTESIAN_POINT ( 'NONE',  ( -16.38289931662955823, -276.6070554962078631, -340.3407213445818229 ) ) ;
#40881=CARTESIAN_POINT ( 'NONE',  ( -95.34786471575526434, -297.8992183611205178, -317.6603497505437304 ) ) ;
#40882=CARTESIAN_POINT ( 'NONE',  ( -46.93527959788583104, -283.9300092129055315, -196.0932234165706802 ) ) ;
#40883=CARTESIAN_POINT ( 'NONE',  ( -27.84748908710411186, -291.8361515741199241, -193.9163312745061205 ) ) ;
#40884=CARTESIAN_POINT ( 'NONE',  ( 36.65426344356991706, -273.4455615773345016, -260.5405183295529241 ) ) ;
#40885=CARTESIAN_POINT ( 'NONE',  ( 9.749716255935902964, -290.0166980007785469, -330.3351778715236833 ) ) ;
#40886=CARTESIAN_POINT ( 'NONE',  ( -34.83299178285379583, -291.0047313505910438, -197.0949425890030113 ) ) ;
#40888=CARTESIAN_POINT ( 'NONE',  ( -19.50655331740970055, -290.8517849429848638, -196.0065514991878786 ) ) ;
#40889=CARTESIAN_POINT ( 'NONE',  ( -109.9934992487361285, -290.3156030965975560, -263.0260262131951094 ) ) ;
#40891=CARTESIAN_POINT ( 'NONE',  ( 25.28470490797628401, -288.0434057776815280, -226.0730789246693178 ) ) ;
#40892=CARTESIAN_POINT ( 'NONE',  ( -108.7845816817346787, -278.6863013625263079, -285.4608584497309494 ) ) ;
#40893=CARTESIAN_POINT ( 'NONE',  ( -64.17097843709920824, -294.3144674217803640, -342.2059670324316585 ) ) ;
#40894=CARTESIAN_POINT ( 'NONE',  ( -91.83661099625958002, -285.9507757439558304, -216.1060032382476379 ) ) ;
#40895=CARTESIAN_POINT ( 'NONE',  ( -0.9832920331938328484, -286.8546714922085243, -202.5097329386007630 ) ) ;
#40896=CARTESIAN_POINT ( 'NONE',  ( 11.93408240144392529, -282.6776104189459602, -324.2497507617106294 ) ) ;
#40897=CARTESIAN_POINT ( 'NONE',  ( 153.7078430325209126, 207.1860052592516013, -217.3454689461144653 ) ) ;
#40898=CARTESIAN_POINT ( 'NONE',  ( 183.8342670656734015, 263.4819769339147797, -152.6844725691555595 ) ) ;
#40899=CARTESIAN_POINT ( 'NONE',  ( 183.6787524270977485, 261.1293638455505857, -151.0742354505036360 ) ) ;
#40900=CARTESIAN_POINT ( 'NONE',  ( 0.7051506998533149106, -273.7708687721664091, -207.8708077817659614 ) ) ;
#40901=CARTESIAN_POINT ( 'NONE',  ( 32.38797661390856319, -274.7714208734319072, -292.9884964230134869 ) ) ;
#40902=CARTESIAN_POINT ( 'NONE',  ( -107.7142036935486402, -296.4584093970260597, -239.1289756098501016 ) ) ;
#40903=CARTESIAN_POINT ( 'NONE',  ( 66.18494971993401066, 45.90398865963478414, -315.9893126914129766 ) ) ;
#40904=CARTESIAN_POINT ( 'NONE',  ( 39.06291576992948222, -274.1756417347864954, -265.4879876495817257 ) ) ;
#40905=CARTESIAN_POINT ( 'NONE',  ( -54.46746588770982100, -275.5892481486159795, -198.3563809298433682 ) ) ;
#40907=CARTESIAN_POINT ( 'NONE',  ( -34.07149460053084056, -299.0334027112224362, -193.5959021688697135 ) ) ;
#40908=CARTESIAN_POINT ( 'NONE',  ( -21.10957504857951506, -289.3305628936617495, -341.5966888503347150 ) ) ;
#40909=CARTESIAN_POINT ( 'NONE',  ( -96.38077122379498007, -296.6918863268394944, -319.5602973641422295 ) ) ;
#40910=CARTESIAN_POINT ( 'NONE',  ( -108.8337426737351450, -297.4070671079502404, -241.7852827642537079 ) ) ;
#40911=CARTESIAN_POINT ( 'NONE',  ( 34.71360014120221393, -293.5633785683979795, -258.5768258089188976 ) ) ;
#40913=CARTESIAN_POINT ( 'NONE',  ( 26.44655563262336884, -278.0143258023581438, -310.9599378445709590 ) ) ;
#40915=CARTESIAN_POINT ( 'NONE',  ( 36.92725390009606912, -280.8074373718260972, -250.2201139663033302 ) ) ;
#40916=CARTESIAN_POINT ( 'NONE',  ( -37.79923683419279001, -277.9992392846198754, -343.6074770607820597 ) ) ;
#40917=CARTESIAN_POINT ( 'NONE',  ( 20.96763879468937830, -277.9766797861123564, -319.0847776445557997 ) ) ;
#40919=CARTESIAN_POINT ( 'NONE',  ( -98.33364197106298832, -275.9720951254918759, -314.6367673584895783 ) ) ;
#40920=CARTESIAN_POINT ( 'NONE',  ( -104.8595255667243720, -297.5788169953463012, -242.3390567462739966 ) ) ;
#40921=CARTESIAN_POINT ( 'NONE',  ( -109.8533898197255212, -295.2910675836055816, -257.8140156865094355 ) ) ;
#40923=CARTESIAN_POINT ( 'NONE',  ( 19.11074369088685287, -281.3318379090331973, -218.0863775229832697 ) ) ;
#40924=CARTESIAN_POINT ( 'NONE',  ( -109.9663383702328900, -278.8227569530467349, -262.4831275639624550 ) ) ;
#40925=CARTESIAN_POINT ( 'NONE',  ( -4.559655801269173914, -287.3140747464676679, -339.5031807684796945 ) ) ;
#40926=CARTESIAN_POINT ( 'NONE',  ( 72.99834851041279649, -301.4305609889117932, -195.1569263972049271 ) ) ;
#40928=CARTESIAN_POINT ( 'NONE',  ( -31.86945840514198736, -288.1786415660986904, -343.3683901364825601 ) ) ;
#40930=CARTESIAN_POINT ( 'NONE',  ( -41.08026103079195934, -278.2443110747364017, -196.4422626262946494 ) ) ;
#40931=CARTESIAN_POINT ( 'NONE',  ( -57.25536489884444080, -278.3648203012128874, -199.5174812106892546 ) ) ;
#40932=CARTESIAN_POINT ( 'NONE',  ( -13.08274929604248982, -280.8144953876131922, -340.7920297080265186 ) ) ;
#40933=CARTESIAN_POINT ( 'NONE',  ( -95.42566117404476245, -287.2063707370795100, -222.8938104063183516 ) ) ;
#40934=CARTESIAN_POINT ( 'NONE',  ( -100.9191528787679175, -279.2558515195320865, -307.1379167346669874 ) ) ;
#40936=CARTESIAN_POINT ( 'NONE',  ( -61.08034301192003568, -293.7442956298834247, -199.1623514990029662 ) ) ;
#40937=CARTESIAN_POINT ( 'NONE',  ( -110.8529042008521373, -276.5474198098099805, -289.6496863254466234 ) ) ;
#40938=CARTESIAN_POINT ( 'NONE',  ( -6.225714457559289983, -277.2836039704966424, -336.5238907322673185 ) ) ;
#40939=CARTESIAN_POINT ( 'NONE',  ( -38.67389111183416617, -285.0689823418150013, -345.5159827458489872 ) ) ;
#40940=CARTESIAN_POINT ( 'NONE',  ( 115.2940338803257703, -299.5541904835127980, -197.7520877843884080 ) ) ;
#40941=CARTESIAN_POINT ( 'NONE',  ( -81.98185092125250151, -291.5755395712980089, -331.3248049816650678 ) ) ;
#40942=CARTESIAN_POINT ( 'NONE',  ( -25.84630414365701867, -292.9057046909653650, -344.5266118690907433 ) ) ;
#40943=CARTESIAN_POINT ( 'NONE',  ( 34.91711868069736369, -287.0817747895744674, -296.6467246737050800 ) ) ;
#40944=CARTESIAN_POINT ( 'NONE',  ( -32.64288430324890555, -272.7974008908149699, -197.0057187629735722 ) ) ;
#40945=CARTESIAN_POINT ( 'NONE',  ( -6.269110277569869716, -292.7790882332398041, -337.7804004123926802 ) ) ;
#40947=CARTESIAN_POINT ( 'NONE',  ( -110.5613795317854198, -289.3039673646861161, -248.8765583812391640 ) ) ;
#40948=CARTESIAN_POINT ( 'NONE',  ( -67.89732362602889282, -287.2443398007634414, -203.1837833389752461 ) ) ;
#40949=CARTESIAN_POINT ( 'NONE',  ( 23.06963481109530534, -285.1691033680874625, -224.2480786117171192 ) ) ;
#40951=CARTESIAN_POINT ( 'NONE',  ( -67.80807798851924417, -287.0695119959246995, -203.3747407199194868 ) ) ;
#40953=CARTESIAN_POINT ( 'NONE',  ( -99.75239657253662529, -285.8810234999037903, -232.0872675049267855 ) ) ;
#40954=CARTESIAN_POINT ( 'NONE',  ( 35.81886551686887543, -295.3012588055818242, -252.3073526920058782 ) ) ;
#40955=CARTESIAN_POINT ( 'NONE',  ( 20.61017094222211909, -274.2969797833857797, -318.8471452555712631 ) ) ;
#40956=CARTESIAN_POINT ( 'NONE',  ( -7.888799347717783128, -277.0099541260258320, -341.4969213389408083 ) ) ;
#40957=CARTESIAN_POINT ( 'NONE',  ( -55.81265611667642190, -289.8961427098901140, -197.0396244884203725 ) ) ;
#40958=CARTESIAN_POINT ( 'NONE',  ( -112.4017312731608058, -278.7669533499513932, -253.1857948560594025 ) ) ;
#40959=CARTESIAN_POINT ( 'NONE',  ( -45.24026552476296104, -297.1324474610444213, -344.6384646975732835 ) ) ;
#40962=CARTESIAN_POINT ( 'NONE',  ( 19.90984047221398967, -285.5896422434225315, -224.2596743818670575 ) ) ;
#40963=CARTESIAN_POINT ( 'NONE',  ( 20.95224922324841188, -280.2018833336271086, -317.5705241888700243 ) ) ;
#40965=CARTESIAN_POINT ( 'NONE',  ( -7.939669693597882549, -272.9101739149491550, -199.8903344400839899 ) ) ;
#40966=CARTESIAN_POINT ( 'NONE',  ( -87.17106446520546115, -277.1174833406175253, -323.8487531678294431 ) ) ;
#40967=CARTESIAN_POINT ( 'NONE',  ( -8.946001522705490316, -296.1940125716217835, -338.3777375388956443 ) ) ;
#40968=CARTESIAN_POINT ( 'NONE',  ( -2.518167510610716420, -279.4221533293300013, -202.0177275191922774 ) ) ;
#40969=CARTESIAN_POINT ( 'NONE',  ( -69.81766495532748706, -296.4319807206471182, -336.0019601270143994 ) ) ;
#40970=EDGE_CURVE ( 'NONE', #92001, #49115, #93363, .T. ) ;
#40971=CARTESIAN_POINT ( 'NONE',  ( -106.7121327851724573, -297.4517027104175781, -302.6262902956850667 ) ) ;
#40972=CARTESIAN_POINT ( 'NONE',  ( -106.3249697826862672, -272.5372377173292193, -246.4154295500165688 ) ) ;
#40973=CARTESIAN_POINT ( 'NONE',  ( -27.87857319862299477, -294.1723383268938505, -195.9083763871365989 ) ) ;
#40974=CARTESIAN_POINT ( 'NONE',  ( -36.56756391987610755, -286.2282954959094354, -193.3519706163582441 ) ) ;
#40975=CARTESIAN_POINT ( 'NONE',  ( 38.14775023160404288, -273.7737627613824429, -276.8146722799290274 ) ) ;
#40976=CARTESIAN_POINT ( 'NONE',  ( 36.38478081270785935, -287.6647871430372447, -292.6196524667047356 ) ) ;
#40977=CARTESIAN_POINT ( 'NONE',  ( -111.8011020342518833, -280.5998799454968093, -265.1033363045849569 ) ) ;
#40978=CARTESIAN_POINT ( 'NONE',  ( 26.57858354566873871, -286.1223175304125448, -234.5137189545126262 ) ) ;
#40979=CARTESIAN_POINT ( 'NONE',  ( -107.5913298006977215, -288.8947816867756728, -243.9455879633486006 ) ) ;
#40980=CARTESIAN_POINT ( 'NONE',  ( -33.93809357080956346, -124.0300793293349244, -358.8670080828285336 ) ) ;
#40981=CARTESIAN_POINT ( 'NONE',  ( 28.86836508021439940, -286.6430427303849342, -239.4707358779378694 ) ) ;
#40984=CARTESIAN_POINT ( 'NONE',  ( 26.53277250174978619, -283.0555388229089999, -312.9389521118226298 ) ) ;
#40985=CARTESIAN_POINT ( 'NONE',  ( -70.78434638461257578, -290.6804907733452410, -201.2640151084531226 ) ) ;
#40986=CARTESIAN_POINT ( 'NONE',  ( -6.572284064420578886, -282.0495870283688760, -200.6355662389266854 ) ) ;
#40987=CARTESIAN_POINT ( 'NONE',  ( 38.69071129616798999, -282.7544173024307952, -261.3910481009908722 ) ) ;
#40988=CARTESIAN_POINT ( 'NONE',  ( 35.68742566989009646, -281.3620502239274401, -268.5856944877209571 ) ) ;
#40989=CARTESIAN_POINT ( 'NONE',  ( -84.18520332195230083, -295.6759877703877919, -331.5404225690522253 ) ) ;
#40990=CARTESIAN_POINT ( 'NONE',  ( -111.0471424113618042, -288.4189246737976191, -282.2465348646594521 ) ) ;
#40991=CARTESIAN_POINT ( 'NONE',  ( -35.12226306307413637, -297.0009042531316368, -197.0524225634412403 ) ) ;
#40994=CARTESIAN_POINT ( 'NONE',  ( -111.5289138776900302, -286.3930167990264977, -276.4906784917459390 ) ) ;
#40995=CARTESIAN_POINT ( 'NONE',  ( 38.93116929254586722, -294.7383758919842194, -278.8469501064081442 ) ) ;
#40996=CARTESIAN_POINT ( 'NONE',  ( 3.453974984907793200, -283.1392718720291555, -331.0821056064041272 ) ) ;
#40997=CARTESIAN_POINT ( 'NONE',  ( -66.12783175073917619, -272.7432462658574082, -199.1839481271519503 ) ) ;
#40998=CARTESIAN_POINT ( 'NONE',  ( -77.12364163750277157, -292.1855127121544911, -204.4915740136052875 ) ) ;
#40999=CARTESIAN_POINT ( 'NONE',  ( -98.33552481205525453, -283.2996234009774525, -225.3297643827825141 ) ) ;
#41000=CARTESIAN_POINT ( 'NONE',  ( 20.36002676216346075, -293.1950654803507632, -219.3877453523765837 ) ) ;
#41001=CARTESIAN_POINT ( 'NONE',  ( 25.71645034331005419, -288.3918729451954732, -307.2816975188655420 ) ) ;
#41004=CARTESIAN_POINT ( 'NONE',  ( -111.0017296283295707, -270.8980037439225157, -283.6562794664417879 ) ) ;
#41005=CARTESIAN_POINT ( 'NONE',  ( -58.27776522270531956, -284.8379308715856837, -343.7945080851740158 ) ) ;
#41006=CARTESIAN_POINT ( 'NONE',  ( -95.95921662488163406, -282.6952119285918457, -223.5744983911110353 ) ) ;
#41008=CARTESIAN_POINT ( 'NONE',  ( 35.87395248041093510, -280.5210855256756304, -274.0616971121617098 ) ) ;
#41009=CARTESIAN_POINT ( 'NONE',  ( -38.54888472703695612, -276.7336221989515366, -347.3305079826367887 ) ) ;
#41010=CARTESIAN_POINT ( 'NONE',  ( -109.3901680170536252, -280.8136479791787110, -250.0886624119323471 ) ) ;
#41011=CARTESIAN_POINT ( 'NONE',  ( 204.5909265758118067, 292.7456558654929495, -53.99999999999697309 ) ) ;
#41012=CARTESIAN_POINT ( 'NONE',  ( -11.68993548917152658, -278.9543417305906701, -198.3292203697543812 ) ) ;
#41013=CARTESIAN_POINT ( 'NONE',  ( -109.3544814497171558, -282.3178547304559629, -290.0564759326584863 ) ) ;
#41014=CARTESIAN_POINT ( 'NONE',  ( -62.53055105828439508, -299.4889568815985399, -198.6708410858421132 ) ) ;
#41015=CARTESIAN_POINT ( 'NONE',  ( 23.38891612813890220, -293.4808946815847435, -229.7436255584644300 ) ) ;
#41017=CARTESIAN_POINT ( 'NONE',  ( -49.75565389035584474, -290.5754591043964865, -197.8723210307584850 ) ) ;
#41018=CARTESIAN_POINT ( 'NONE',  ( 14.82013526042823592, -276.9917270619812939, -326.9354187106717404 ) ) ;
#41019=CARTESIAN_POINT ( 'NONE',  ( -36.73606981722915776, -274.0599701988010111, -197.3512152546650213 ) ) ;
#41020=CARTESIAN_POINT ( 'NONE',  ( -76.26393811409228363, -272.4653375313710626, -204.2198718604255419 ) ) ;
#41022=CARTESIAN_POINT ( 'NONE',  ( 17.83788013527916050, -272.8415312382531397, -219.4908323982217269 ) ) ;
#41024=CARTESIAN_POINT ( 'NONE',  ( -5.887893459300612697, -283.7083868166416778, -336.5933850397269680 ) ) ;
#41025=CARTESIAN_POINT ( 'NONE',  ( 34.36389418194562495, -282.9891025477809308, -245.0588858332488655 ) ) ;
#41026=CARTESIAN_POINT ( 'NONE',  ( -109.2918805855209712, -284.0719324168400135, -257.3654096347033260 ) ) ;
#41027=CARTESIAN_POINT ( 'NONE',  ( 27.34747739560153690, -273.4708344689531714, -234.7334258174505237 ) ) ;
#41028=CARTESIAN_POINT ( 'NONE',  ( -19.25618201513518102, -282.1476046482051174, -198.3094791408386754 ) ) ;
#41029=CARTESIAN_POINT ( 'NONE',  ( 34.18677836911302137, -273.8002544740293729, -252.6302263465097724 ) ) ;
#41031=CARTESIAN_POINT ( 'NONE',  ( 35.89498921751919625, -276.5759526496502758, -266.1073878607876964 ) ) ;
#41033=CARTESIAN_POINT ( 'NONE',  ( -74.93786875106941636, -280.3673766076088327, -203.3485301688253344 ) ) ;
#41035=EDGE_LOOP ( 'NONE', ( #85380, #47066, #42042, #16919 ) ) ;
#41037=CARTESIAN_POINT ( 'NONE',  ( -112.2695581055860004, -286.5597132902533417, -258.7840618111244453 ) ) ;
#41038=CARTESIAN_POINT ( 'NONE',  ( -18.18804956194439626, -293.9960510009242967, -340.9708864035305282 ) ) ;
#41039=CARTESIAN_POINT ( 'NONE',  ( -89.42853896968865968, -289.1118691119034452, -326.9320823178122168 ) ) ;
#41041=CARTESIAN_POINT ( 'NONE',  ( -27.68241467193774596, -284.4163637195857746, -196.9807921682487972 ) ) ;
#41042=CARTESIAN_POINT ( 'NONE',  ( 17.34052456815976129, -285.4272333429417472, -221.0956838386867105 ) ) ;
#41043=CARTESIAN_POINT ( 'NONE',  ( -20.92609229013621785, -287.0784369559788161, -342.5310690022453741 ) ) ;
#41044=CARTESIAN_POINT ( 'NONE',  ( -87.18730424682998148, -284.9701123275049781, -324.3059212820268158 ) ) ;
#41045=CARTESIAN_POINT ( 'NONE',  ( 34.56841783194239781, -273.8269462204076490, -291.7121402763479523 ) ) ;
#41047=CARTESIAN_POINT ( 'NONE',  ( 37.24469658391227966, -285.7541029660586105, -254.6994679130625343 ) ) ;
#41048=CARTESIAN_POINT ( 'NONE',  ( -95.80380541415016182, -299.1986782225042703, -223.3804528207505768 ) ) ;
#41049=CARTESIAN_POINT ( 'NONE',  ( 37.51923030184178032, -285.6387572784083204, -277.1338220136053678 ) ) ;
#41051=CARTESIAN_POINT ( 'NONE',  ( -32.96087733198928049, -281.0499519129303394, -197.2569673476132266 ) ) ;
#41052=CARTESIAN_POINT ( 'NONE',  ( -74.72914985887028649, -291.5487809407809436, -335.5700669834781706 ) ) ;
#41055=CARTESIAN_POINT ( 'NONE',  ( -70.15990221002310534, -297.4012268675285213, -338.4362087182920504 ) ) ;
#41057=CARTESIAN_POINT ( 'NONE',  ( -4.664704406898105837, -278.4824537590569093, -202.8539731433333770 ) ) ;
#41058=CARTESIAN_POINT ( 'NONE',  ( 32.04455791834918443, -292.3239142321250483, -237.2267358849973675 ) ) ;
#41059=CARTESIAN_POINT ( 'NONE',  ( -100.5718153847858787, -295.4711962084401762, -232.2040246678462267 ) ) ;
#41060=CARTESIAN_POINT ( 'NONE',  ( 13.68950125206323243, -279.4699642856195396, -217.4029444286035471 ) ) ;
#41061=CARTESIAN_POINT ( 'NONE',  ( -51.81801856788109006, -271.9454752426740924, -197.2894743900849619 ) ) ;
#41062=CARTESIAN_POINT ( 'NONE',  ( 18.35705956718997101, -295.5457357073779576, -318.3270702093866475 ) ) ;
#41063=CARTESIAN_POINT ( 'NONE',  ( 10.59707575819634329, -289.1948066931273615, -210.1954327657594490 ) ) ;
#41064=CARTESIAN_POINT ( 'NONE',  ( -86.99628088328472586, -295.8556977659026757, -212.3507284482672048 ) ) ;
#41065=CARTESIAN_POINT ( 'NONE',  ( -55.91906201822835953, -290.0561298046563934, -196.6261291310442800 ) ) ;
#41067=CARTESIAN_POINT ( 'NONE',  ( -77.59249977129567810, -292.9254054567558683, -208.7555334598870900 ) ) ;
#41069=CARTESIAN_POINT ( 'NONE',  ( -108.2675357336823794, -291.5919497537067286, -252.3622252116168170 ) ) ;
#41071=CARTESIAN_POINT ( 'NONE',  ( -89.21128656762166997, -290.9680590858306459, -326.7309212488149228 ) ) ;
#41072=CARTESIAN_POINT ( 'NONE',  ( 21.22856885401114013, -280.2221483384781209, -317.7938120302768539 ) ) ;
#41073=CARTESIAN_POINT ( 'NONE',  ( 34.83797523761040082, -293.7004506830211881, -281.6029558478151671 ) ) ;
#41074=CARTESIAN_POINT ( 'NONE',  ( -4.943987858190243223, -280.4670622808420717, -200.5084999952766509 ) ) ;
#41075=CARTESIAN_POINT ( 'NONE',  ( -90.42663185398420467, -283.4455469431989059, -326.1812675011128704 ) ) ;
#41076=CARTESIAN_POINT ( 'NONE',  ( -96.41308611418976682, -287.9203992113521622, -316.3230952909382836 ) ) ;
#41077=CARTESIAN_POINT ( 'NONE',  ( -109.9328245700958604, -282.4894047668310009, -285.9584448127796463 ) ) ;
#41079=CARTESIAN_POINT ( 'NONE',  ( 18.66455657022052605, -279.3196935458660164, -218.5344167227259504 ) ) ;
#41080=CARTESIAN_POINT ( 'NONE',  ( 0.1447540201736723098, -285.4594398357559726, -203.4412846360525577 ) ) ;
#41082=CARTESIAN_POINT ( 'NONE',  ( 22.44092148809162168, -294.5531993029314322, -227.0674906946891269 ) ) ;
#41083=CARTESIAN_POINT ( 'NONE',  ( -59.47684553821569864, -278.7585819558410662, -343.4955259535610708 ) ) ;
#41084=CARTESIAN_POINT ( 'NONE',  ( -72.85600040899018381, -277.2031654759853723, -334.1784976719630436 ) ) ;
#41085=CARTESIAN_POINT ( 'NONE',  ( -114.1122943306870496, -290.6363573704136343, -276.9557053438076650 ) ) ;
#41086=CARTESIAN_POINT ( 'NONE',  ( -44.31121230131459043, -281.2193612437335446, -345.6513683574550555 ) ) ;
#41087=CARTESIAN_POINT ( 'NONE',  ( 21.50841941490298126, -293.2201259787927938, -313.9509319124732656 ) ) ;
#41088=CARTESIAN_POINT ( 'NONE',  ( -110.3221715027138998, -294.7739764965101017, -253.0737974500453902 ) ) ;
#41090=CARTESIAN_POINT ( 'NONE',  ( 28.44723814067911505, -293.4908881261306419, -302.2551843027393943 ) ) ;
#41092=CARTESIAN_POINT ( 'NONE',  ( -105.5937364680635966, -281.8380690714489560, -285.9065529553535612 ) ) ;
#41093=CARTESIAN_POINT ( 'NONE',  ( -106.9580446188182918, -295.1956398645567106, -302.7089895049489314 ) ) ;
#41094=CARTESIAN_POINT ( 'NONE',  ( 33.18347853754416832, -279.3334083564326988, -242.5319898106522487 ) ) ;
#41095=CARTESIAN_POINT ( 'NONE',  ( -37.99514509914298799, -287.3592933896689487, -193.8570574067196048 ) ) ;
#41096=CARTESIAN_POINT ( 'NONE',  ( -14.56398944898162995, -286.1889561105984967, -200.9526672256791642 ) ) ;
#41097=CARTESIAN_POINT ( 'NONE',  ( -87.55393819312332937, -279.2886687997292370, -324.3003328419721356 ) ) ;
#41098=CARTESIAN_POINT ( 'NONE',  ( -96.08307975919393584, -293.9371522448985843, -316.4186594490874995 ) ) ;
#41099=CARTESIAN_POINT ( 'NONE',  ( -109.8733455967555983, -298.1197511453075322, -285.1596232922974536 ) ) ;
#41100=CARTESIAN_POINT ( 'NONE',  ( -74.22601906662013960, -276.3491885353718089, -333.8172250289101157 ) ) ;
#41102=CARTESIAN_POINT ( 'NONE',  ( -102.2962767623809981, -296.7605036603702047, -229.0495304344446765 ) ) ;
#41103=CARTESIAN_POINT ( 'NONE',  ( -76.60797044999216610, -291.5022224941862987, -333.6025143307660414 ) ) ;
#41104=CARTESIAN_POINT ( 'NONE',  ( 20.77089707463454360, -295.8236021285290462, -319.6497217736782090 ) ) ;
#41105=CARTESIAN_POINT ( 'NONE',  ( 201.7545824283169225, 292.3729076405792284, -53.99999999997594813 ) ) ;
#41106=CARTESIAN_POINT ( 'NONE',  ( 27.12426616765833032, -288.6740425020491898, -304.9367141524379008 ) ) ;
#41108=CARTESIAN_POINT ( 'NONE',  ( 24.05966901727094864, -281.2260032550470328, -316.4338005692189881 ) ) ;
#41109=CARTESIAN_POINT ( 'NONE',  ( -111.8678020810175013, -296.9654994036794733, -289.3661116125622925 ) ) ;
#41110=CARTESIAN_POINT ( 'NONE',  ( -110.0401751519187883, -288.9637283464268762, -249.0248293968679718 ) ) ;
#41111=CARTESIAN_POINT ( 'NONE',  ( -70.72371292266220166, -297.9571016812775497, -200.9969664814844066 ) ) ;
#41116=CARTESIAN_POINT ( 'NONE',  ( 16.21326865916951476, -289.8292784396544448, -324.7905985224219876 ) ) ;
#41117=CARTESIAN_POINT ( 'NONE',  ( -115.3288506153726871, -294.2666405000204009, -252.5284128619063608 ) ) ;
#41119=CARTESIAN_POINT ( 'NONE',  ( 34.23259412519036715, -280.5422164157160410, -242.1010992490742808 ) ) ;
#41120=CARTESIAN_POINT ( 'NONE',  ( -110.4615939364114183, -286.7579729771636607, -254.3792174287803789 ) ) ;
#41121=CARTESIAN_POINT ( 'NONE',  ( 37.52728857025744702, -286.3193587878362223, -285.6333419849396478 ) ) ;
#41122=CARTESIAN_POINT ( 'NONE',  ( 1.587401756308150835, -272.5737339517414171, -206.4506066993375271 ) ) ;
#41123=CARTESIAN_POINT ( 'NONE',  ( -107.6747952551809817, -274.7903097030651338, -245.9773133815993447 ) ) ;
#41124=VECTOR ( 'NONE', #12343, 1000.000000000000000 ) ;
#41125=CARTESIAN_POINT ( 'NONE',  ( -103.6820029439865749, -289.0831070532123590, -236.4790781022847739 ) ) ;
#41126=CARTESIAN_POINT ( 'NONE',  ( -113.1486265574077947, -280.3966697992362924, -271.6120325674877449 ) ) ;
#41127=CARTESIAN_POINT ( 'NONE',  ( -7.999445884722894640, -280.4475527640443602, -203.5041054592432488 ) ) ;
#41128=CARTESIAN_POINT ( 'NONE',  ( 34.03815350793523464, -281.1085283059636026, -286.1348037747450803 ) ) ;
#41129=CARTESIAN_POINT ( 'NONE',  ( -28.62247023842397553, -278.0238402580508250, -346.6080977672831409 ) ) ;
#41130=CARTESIAN_POINT ( 'NONE',  ( -45.21720561371426328, -278.7495688390453665, -194.1113859238821249 ) ) ;
#41131=CARTESIAN_POINT ( 'NONE',  ( 159.2613953296296643, 219.3517484348739401, -203.0981120538807545 ) ) ;
#41132=CARTESIAN_POINT ( 'NONE',  ( -94.91796165021136744, -274.1829569011866852, -219.5891343453561433 ) ) ;
#41133=EDGE_CURVE ( 'NONE', #25769, #81416, #14413, .T. ) ;
#41134=CARTESIAN_POINT ( 'NONE',  ( -109.4530370487537283, -274.3897128112149062, -245.4079049736626246 ) ) ;
#41135=CARTESIAN_POINT ( 'NONE',  ( 31.98288692825981272, -290.4805209788416391, -303.7098442033569654 ) ) ;
#41138=CARTESIAN_POINT ( 'NONE',  ( 35.98918607386463719, -288.6046246368758261, -268.2900672227270320 ) ) ;
#41139=CARTESIAN_POINT ( 'NONE',  ( 32.91385123181829186, -288.9379057052419171, -241.2732564096131682 ) ) ;
#41140=CARTESIAN_POINT ( 'NONE',  ( -50.77832957252943658, -288.5768004351575655, -342.2693218052381212 ) ) ;
#41141=CARTESIAN_POINT ( 'NONE',  ( -104.3664900499624082, -283.5679844076287281, -308.2473987396795678 ) ) ;
#41142=CARTESIAN_POINT ( 'NONE',  ( 19.46480550931818954, -279.2909681565450910, -223.2303382217800163 ) ) ;
#41143=CARTESIAN_POINT ( 'NONE',  ( -71.77179245318097855, -287.4524536214564137, -204.5930845234890967 ) ) ;
#41144=CARTESIAN_POINT ( 'NONE',  ( 36.39632857189117487, -280.0448416946348971, -271.3421247772542984 ) ) ;
#41145=CARTESIAN_POINT ( 'NONE',  ( -98.41268100256962725, -280.4324349415506390, -229.3857787574259817 ) ) ;
#41146=CARTESIAN_POINT ( 'NONE',  ( -35.10947924728646541, -277.5157167606794815, -343.3885486628410604 ) ) ;
#41147=CARTESIAN_POINT ( 'NONE',  ( -89.23382792912653372, -288.5582957521842786, -326.7101711242518718 ) ) ;
#41148=CARTESIAN_POINT ( 'NONE',  ( -102.7752060292336296, -284.8273778980123438, -310.6428151376581468 ) ) ;
#41149=CARTESIAN_POINT ( 'NONE',  ( -74.24095428152287468, -284.0211171267319514, -337.9333141188182026 ) ) ;
#41150=CARTESIAN_POINT ( 'NONE',  ( -29.44254347037384179, -283.1161327696497665, -342.9829888053851050 ) ) ;
#41153=CARTESIAN_POINT ( 'NONE',  ( -97.16941640809957903, -291.7815902524616831, -316.8471357616768955 ) ) ;
#41154=CARTESIAN_POINT ( 'NONE',  ( 20.94568398526683595, -291.5643690565316888, -220.7842708659962625 ) ) ;
#41155=CARTESIAN_POINT ( 'NONE',  ( -3.986854391651197371, -273.5620172079876511, -205.1483984843130770 ) ) ;
#41156=CARTESIAN_POINT ( 'NONE',  ( -97.33313446893353671, -295.2551120485818501, -318.4895539335668673 ) ) ;
#41157=CARTESIAN_POINT ( 'NONE',  ( -17.22490996144808406, -290.7962931388438506, -199.4135753120056336 ) ) ;
#41158=CARTESIAN_POINT ( 'NONE',  ( -5.120342306461822091, -292.8619564273380433, -337.0066277221436621 ) ) ;
#41159=CARTESIAN_POINT ( 'NONE',  ( -99.16802386047204720, -291.2130351277514251, -309.9166005146893212 ) ) ;
#41161=CARTESIAN_POINT ( 'NONE',  ( -110.3107676467127050, -292.3290191752894884, -287.7513845534626284 ) ) ;
#41162=CARTESIAN_POINT ( 'NONE',  ( -34.99159093599732984, -290.0814155835148540, -195.2183576876095970 ) ) ;
#41163=CARTESIAN_POINT ( 'NONE',  ( -71.42834417707278760, -297.5024156777060398, -337.1817468121076899 ) ) ;
#41164=CARTESIAN_POINT ( 'NONE',  ( 18.83455950827622161, -287.8284171611957731, -223.3560945960349784 ) ) ;
#41165=CARTESIAN_POINT ( 'NONE',  ( -11.65908633609343426, -296.7187942262509637, -341.0593362159445405 ) ) ;
#41166=CARTESIAN_POINT ( 'NONE',  ( 10.71689283427927819, -276.6920719183102619, -212.2521525024003779 ) ) ;
#41167=CARTESIAN_POINT ( 'NONE',  ( 98.84066493780467511, -298.9135927194789701, -193.5404977642008930 ) ) ;
#41168=CARTESIAN_POINT ( 'NONE',  ( 5.971903607451601204, -274.6959184177126758, -330.4402727933716619 ) ) ;
#41169=CARTESIAN_POINT ( 'NONE',  ( -62.77847166040100291, -277.7984397897478175, -200.3475505220830541 ) ) ;
#41170=CARTESIAN_POINT ( 'NONE',  ( -35.14592078867098479, -299.3953797982574088, -196.8674597293335466 ) ) ;
#41171=CARTESIAN_POINT ( 'NONE',  ( 23.17736608043865587, -273.4993226203873746, -223.6916750528299076 ) ) ;
#41172=CARTESIAN_POINT ( 'NONE',  ( -68.75248953991011547, -296.8985641019899049, -336.9237171196394911 ) ) ;
#41174=CARTESIAN_POINT ( 'NONE',  ( -107.7554486521644037, -297.0930039502329123, -290.2232866971413046 ) ) ;
#41177=CARTESIAN_POINT ( 'NONE',  ( -26.40864434976349884, -286.9337763603784879, -344.9189820346633724 ) ) ;
#41178=CARTESIAN_POINT ( 'NONE',  ( -92.01675149714054669, -273.0765498590686775, -221.9913054719793877 ) ) ;
#41180=CARTESIAN_POINT ( 'NONE',  ( -49.34472809488563882, -285.9033314182544814, -194.2486724588901836 ) ) ;
#41181=CARTESIAN_POINT ( 'NONE',  ( -82.84356402013463594, -289.3224670658993318, -332.4523788313267687 ) ) ;
#41182=CARTESIAN_POINT ( 'NONE',  ( -111.9762840897595595, -298.6660994108328282, -259.8711284591287267 ) ) ;
#41183=CARTESIAN_POINT ( 'NONE',  ( -8.548441092542681474, -292.6742987303485961, -339.4473200087999771 ) ) ;
#41185=CARTESIAN_POINT ( 'NONE',  ( 39.45808755723345485, -280.7798951619258787, -272.8006735779704854 ) ) ;
#41186=CARTESIAN_POINT ( 'NONE',  ( -20.19161114001082069, -289.7666405000204577, -195.3683826091709363 ) ) ;
#41188=CARTESIAN_POINT ( 'NONE',  ( 4.254320565826858136, -278.6123115460059125, -207.8917537791145946 ) ) ;
#41190=CARTESIAN_POINT ( 'NONE',  ( 12.41376360154817604, -287.1357938658919693, -324.3887089515143316 ) ) ;
#41193=CARTESIAN_POINT ( 'NONE',  ( -73.34061479046752652, -287.5294987980494739, -336.1568533582429836 ) ) ;
#41194=CARTESIAN_POINT ( 'NONE',  ( -94.24330054535435863, -298.8114375956258186, -223.3451945514177623 ) ) ;
#41195=CARTESIAN_POINT ( 'NONE',  ( 1.807949475871903688, -283.9644313694084303, -335.9805604405766530 ) ) ;
#41196=CARTESIAN_POINT ( 'NONE',  ( -64.91613223996833426, -295.7140085549717128, -200.1764909488042861 ) ) ;
#41197=CARTESIAN_POINT ( 'NONE',  ( 27.78139285383101154, -281.1029593220091556, -237.2644502935618505 ) ) ;
#41198=CARTESIAN_POINT ( 'NONE',  ( -111.2147876921270182, -296.4458546349878247, -292.1278166581992082 ) ) ;
#41199=CARTESIAN_POINT ( 'NONE',  ( -3.852615762558396550, -275.9281586949315965, -204.8194512522468074 ) ) ;
#41201=CARTESIAN_POINT ( 'NONE',  ( -12.20431818888519793, -282.3792223700725685, -199.6446373813822959 ) ) ;
#41202=CARTESIAN_POINT ( 'NONE',  ( -110.6508120073928012, -271.4726545095895744, -270.3474032455676479 ) ) ;
#41203=ORIENTED_EDGE ( 'NONE', *, *, #12372, .F. ) ;
#41204=CARTESIAN_POINT ( 'NONE',  ( 204.7706911773244087, 294.8516371035053680, -54.00000000003474554 ) ) ;
#41205=CARTESIAN_POINT ( 'NONE',  ( -63.15481001598478628, -287.6943202866786464, -200.2664975874406537 ) ) ;
#41206=CARTESIAN_POINT ( 'NONE',  ( 133.0872704186301405, -299.5541904835127980, -195.3611179825600175 ) ) ;
#41207=CARTESIAN_POINT ( 'NONE',  ( 40.65961533371913106, -272.8380690714490129, -252.5904736702033802 ) ) ;
#41208=CARTESIAN_POINT ( 'NONE',  ( -112.6374533610341331, -277.5565052924652605, -285.7463783904381671 ) ) ;
#41209=CARTESIAN_POINT ( 'NONE',  ( -113.2082757868019627, -289.0488828482635881, -262.6969488846294780 ) ) ;
#41210=CARTESIAN_POINT ( 'NONE',  ( -26.62297940217047554, -284.4335973981821439, -343.3225546131592978 ) ) ;
#41211=CARTESIAN_POINT ( 'NONE',  ( 28.56669927013647836, -276.7065000514105009, -237.1568516633402623 ) ) ;
#41212=AXIS2_PLACEMENT_3D ( 'NONE', #57452, #36120, #37049 ) ;
#41213=CARTESIAN_POINT ( 'NONE',  ( -99.29996126232215659, -285.3788704107144554, -315.1684156594441788 ) ) ;
#41214=CARTESIAN_POINT ( 'NONE',  ( -103.3765806782274552, -282.9142958194165658, -302.5173212792527124 ) ) ;
#41215=CARTESIAN_POINT ( 'NONE',  ( -37.02475649072119523, -282.0562785229693645, -195.3617833173209704 ) ) ;
#41216=CARTESIAN_POINT ( 'NONE',  ( -49.72133113237252644, -274.0652513636412095, -194.3089917652966392 ) ) ;
#41217=CARTESIAN_POINT ( 'NONE',  ( -91.33054965403859171, -277.6275420282493087, -325.3375551474478584 ) ) ;
#41218=CARTESIAN_POINT ( 'NONE',  ( -28.70510105053843120, -296.8620878543105732, -344.3504327012894919 ) ) ;
#41221=CARTESIAN_POINT ( 'NONE',  ( -113.0018702431286641, -294.6297757981480459, -275.2359043707697310 ) ) ;
#41222=CARTESIAN_POINT ( 'NONE',  ( 30.33266191769419962, -275.4299375486892245, -298.0305782652033599 ) ) ;
#41223=CARTESIAN_POINT ( 'NONE',  ( -31.95041609189772913, -299.1978304314974366, -193.6692652193777633 ) ) ;
#41224=CARTESIAN_POINT ( 'NONE',  ( -38.66520113531282021, -287.7955088978765161, -196.3469609180639566 ) ) ;
#41225=CARTESIAN_POINT ( 'NONE',  ( -32.04117046317639961, -296.5065739624205889, -346.4966029843527622 ) ) ;
#41226=CARTESIAN_POINT ( 'NONE',  ( 34.08698560629319019, -294.4031349381732525, -242.5387764450289012 ) ) ;
#41227=CARTESIAN_POINT ( 'NONE',  ( -111.2252005397637191, -292.3983347650163864, -282.3266985220449214 ) ) ;
#41228=CARTESIAN_POINT ( 'NONE',  ( 8.279669297338815070, -278.6773768291982947, -210.9767458494015102 ) ) ;
#41229=CARTESIAN_POINT ( 'NONE',  ( -104.6827629162619360, -280.8940871006320208, -238.5145631335620351 ) ) ;
#41230=CARTESIAN_POINT ( 'NONE',  ( -111.1610214454702401, -294.7611161423004091, -260.3798860915666751 ) ) ;
#41231=CARTESIAN_POINT ( 'NONE',  ( -55.38469703066005678, -285.1423157109778685, -343.9461418704025277 ) ) ;
#41232=CARTESIAN_POINT ( 'NONE',  ( -110.6284198035847481, -283.4294252206301508, -273.6383000622860209 ) ) ;
#41233=CARTESIAN_POINT ( 'NONE',  ( 204.9738707124548966, 293.6304025755547968, -68.53118252596463833 ) ) ;
#41235=CARTESIAN_POINT ( 'NONE',  ( -62.56619406408992035, -285.3815198943786982, -201.7811976918543166 ) ) ;
#41237=CARTESIAN_POINT ( 'NONE',  ( 11.30717336774200632, -283.4760513993695668, -329.7154246927971144 ) ) ;
#41238=CARTESIAN_POINT ( 'NONE',  ( -99.30066256563158333, -273.4186113689000308, -231.7195023278788426 ) ) ;
#41239=CARTESIAN_POINT ( 'NONE',  ( 38.96063145376592729, -286.2546751330123129, -263.0107060427403667 ) ) ;
#41240=CARTESIAN_POINT ( 'NONE',  ( 39.40489128974311939, -282.4519348231373215, -267.0555165994222762 ) ) ;
#41241=CARTESIAN_POINT ( 'NONE',  ( -48.37443537269673755, -278.7101166351053507, -345.9194027389390271 ) ) ;
#41242=CARTESIAN_POINT ( 'NONE',  ( -3.709690086294829214, -281.1357149427943227, -201.1931624113720716 ) ) ;
#41243=CARTESIAN_POINT ( 'NONE',  ( -109.1418805571601069, -276.0523547857346784, -270.3284710469131937 ) ) ;
#41244=CARTESIAN_POINT ( 'NONE',  ( 201.0027984253578666, 288.7662968377554193, -97.50545772727659255 ) ) ;
#41247=CARTESIAN_POINT ( 'NONE',  ( -93.40821220137200953, -275.2430403368559837, -220.7972737791770328 ) ) ;
#41248=CARTESIAN_POINT ( 'NONE',  ( 4.936003717816790370, -58.01961007492668898, -354.3995137328890905 ) ) ;
#41250=CARTESIAN_POINT ( 'NONE',  ( -109.8822779568667727, -276.7993404582289827, -252.7624994333112056 ) ) ;
#41251=CARTESIAN_POINT ( 'NONE',  ( 36.76795595612152567, -295.0989027623976995, -253.5179565413668854 ) ) ;
#41252=CARTESIAN_POINT ( 'NONE',  ( -42.40505393370229825, -294.4662792987087983, -343.2874857553237007 ) ) ;
#41253=CARTESIAN_POINT ( 'NONE',  ( -0.8275322185403718445, -292.0314911855879245, -202.6393161368531821 ) ) ;
#41257=CARTESIAN_POINT ( 'NONE',  ( -107.8384937025143415, -294.7475540741158397, -299.9736937379801702 ) ) ;
#41258=CARTESIAN_POINT ( 'NONE',  ( 24.16509862317047919, -286.5121115119811179, -311.1684298047982793 ) ) ;
#41259=CARTESIAN_POINT ( 'NONE',  ( 19.40575695475984475, -294.7438685615165923, -222.5009926431640110 ) ) ;
#41261=CARTESIAN_POINT ( 'NONE',  ( -103.4489830572864548, -285.4341400746934028, -302.5882270590924463 ) ) ;
#41263=CARTESIAN_POINT ( 'NONE',  ( -114.1337742174287229, -291.5183455598047431, -268.3728042826384126 ) ) ;
#41265=CARTESIAN_POINT ( 'NONE',  ( 31.41463957922851336, -282.3750754717723908, -295.2201340125697584 ) ) ;
#41266=CARTESIAN_POINT ( 'NONE',  ( -61.48106938854082415, -294.1536938479402465, -343.1166396591279408 ) ) ;
#41267=CARTESIAN_POINT ( 'NONE',  ( -73.08965571483332724, -290.3165170562892285, -338.3923295689095880 ) ) ;
#41268=CARTESIAN_POINT ( 'NONE',  ( -78.09848545163190181, -290.0764527527808809, -335.6797670342228912 ) ) ;
#41269=CARTESIAN_POINT ( 'NONE',  ( 4.723633750092860240, -286.8043202912064658, -210.6376514534353817 ) ) ;
#41272=CARTESIAN_POINT ( 'NONE',  ( -91.79255679770795950, -297.6790261288470560, -323.0432751886407345 ) ) ;
#41274=CARTESIAN_POINT ( 'NONE',  ( -29.10869328681776835, -296.8380300421357560, -193.8560607233932274 ) ) ;
#41275=CARTESIAN_POINT ( 'NONE',  ( -67.39191009270089694, -278.7068357384384854, -203.5612929295071467 ) ) ;
#41276=CARTESIAN_POINT ( 'NONE',  ( -21.36144848974205601, -273.7594791896040647, -195.1005143400768702 ) ) ;
#41277=CARTESIAN_POINT ( 'NONE',  ( -107.3595220539818911, -295.3360999246783081, -247.2166030724141592 ) ) ;
#41278=CARTESIAN_POINT ( 'NONE',  ( -93.64831600126241540, -279.7352095245564101, -318.7391139244425631 ) ) ;
#41279=CARTESIAN_POINT ( 'NONE',  ( 36.06660057890775306, -273.5472873996151861, -259.2261164537891318 ) ) ;
#41280=CARTESIAN_POINT ( 'NONE',  ( -75.85340846279034110, -296.7835291980024408, -332.9021927488255983 ) ) ;
#41281=CARTESIAN_POINT ( 'NONE',  ( -94.70174383783722760, -298.2737644288790761, -224.7097055140803832 ) ) ;
#41283=CARTESIAN_POINT ( 'NONE',  ( -85.86999987757030794, -297.3117120165575784, -329.1101140322011247 ) ) ;
#41285=CARTESIAN_POINT ( 'NONE',  ( -37.23011418868981792, -296.0533920953740221, -195.1937350554261172 ) ) ;
#41286=CARTESIAN_POINT ( 'NONE',  ( -90.83943233965777608, -291.9190547891043366, -220.5240839346854216 ) ) ;
#41287=CARTESIAN_POINT ( 'NONE',  ( -94.97215231731705387, -274.0445598521916395, -219.5389790939195223 ) ) ;
#41288=CARTESIAN_POINT ( 'NONE',  ( -92.86818249434146821, -288.4431866215342097, -318.7299902590988268 ) ) ;
#41290=CARTESIAN_POINT ( 'NONE',  ( 24.42671822047764252, -275.4340821579542080, -224.4896737266387845 ) ) ;
#41291=CARTESIAN_POINT ( 'NONE',  ( -110.4052107008391204, -296.8708425278252321, -271.4676713260424776 ) ) ;
#41292=CARTESIAN_POINT ( 'NONE',  ( 2.921368067043745853, -282.5691681888419566, -206.6026171118178922 ) ) ;
#41293=CARTESIAN_POINT ( 'NONE',  ( 37.38024129389184225, -280.4445437357587139, -286.8510985108100044 ) ) ;
#41294=CARTESIAN_POINT ( 'NONE',  ( -109.6437641215550514, -277.5678098567039456, -296.7032733476090129 ) ) ;
#41295=CARTESIAN_POINT ( 'NONE',  ( 38.07653713332280887, -280.0896152924329385, -281.2482619475419483 ) ) ;
#41296=CARTESIAN_POINT ( 'NONE',  ( 37.05303910510736642, -279.6896477433839436, -281.1059400452538171 ) ) ;
#41297=CARTESIAN_POINT ( 'NONE',  ( -62.21189748978583367, -272.2969730615606068, -201.1018355722397075 ) ) ;
#41298=CARTESIAN_POINT ( 'NONE',  ( -26.75690723031630824, -278.9178193966616846, -344.6622788111404816 ) ) ;
#41301=CARTESIAN_POINT ( 'NONE',  ( -20.76251538403682417, -296.4968702432226451, -194.3793322445775118 ) ) ;
#41302=CARTESIAN_POINT ( 'NONE',  ( -2.055838212670591858, -292.5062544488460503, -201.9072583069217046 ) ) ;
#41303=CARTESIAN_POINT ( 'NONE',  ( -23.25684604428048630, -278.8727487948989392, -344.2492734776062093 ) ) ;
#41304=CARTESIAN_POINT ( 'NONE',  ( -51.92610362168312577, -271.8654817042391301, -196.7396059933332424 ) ) ;
#41305=CARTESIAN_POINT ( 'NONE',  ( 132.9888089158688445, -299.5541904835127980, -195.3611179825600175 ) ) ;
#41306=CARTESIAN_POINT ( 'NONE',  ( -109.3064616375037303, -286.1767439981734924, -293.4338811728729297 ) ) ;
#41308=CARTESIAN_POINT ( 'NONE',  ( -16.22858399576231037, -286.7791815031728788, -342.3815504752983543 ) ) ;
#41310=CARTESIAN_POINT ( 'NONE',  ( -31.58644725277014231, -293.7729414118836644, -343.5825881740855721 ) ) ;
#41311=CARTESIAN_POINT ( 'NONE',  ( 5.456503627177974991, -284.7775506207781859, -209.6419621142031247 ) ) ;
#41313=CARTESIAN_POINT ( 'NONE',  ( 31.31084012750758561, -291.9474178873009009, -300.5576304016474296 ) ) ;
#41314=CARTESIAN_POINT ( 'NONE',  ( -37.95725395690548254, -284.5244563489983420, -194.0569316687667367 ) ) ;
#41315=CARTESIAN_POINT ( 'NONE',  ( -111.1519674929121209, -280.1843802921181918, -267.9017107689502382 ) ) ;
#41316=CARTESIAN_POINT ( 'NONE',  ( 23.53648252730269519, -288.1338406805382419, -223.8438576788823298 ) ) ;
#41317=CARTESIAN_POINT ( 'NONE',  ( 35.50075884867473519, -280.0691117090692046, -292.1741021061494621 ) ) ;
#41318=CARTESIAN_POINT ( 'NONE',  ( 20.35746322284307652, -288.1821815778940277, -315.1005538123423548 ) ) ;
#41320=CARTESIAN_POINT ( 'NONE',  ( -108.8666207872145151, -280.2039538355605828, -253.0532976802600160 ) ) ;
#41321=CARTESIAN_POINT ( 'NONE',  ( -24.85886971923855171, -281.0183180349987992, -198.2724179561660947 ) ) ;
#41322=CARTESIAN_POINT ( 'NONE',  ( -57.34413665464356313, -287.7753045629299891, -197.6549696322861678 ) ) ;
#41326=CARTESIAN_POINT ( 'NONE',  ( -37.25145703024865895, -297.8865755847954233, -193.3603567442300459 ) ) ;
#41327=CARTESIAN_POINT ( 'NONE',  ( -79.07355589496947346, -291.5975144955892233, -332.3127405254086284 ) ) ;
#41329=CARTESIAN_POINT ( 'NONE',  ( -37.30987171927208124, -291.5519495502701375, -350.3611179825600175 ) ) ;
#41331=CARTESIAN_POINT ( 'NONE',  ( 22.19667473073898378, -272.9245274682088507, -224.4575875660702877 ) ) ;
#41333=CARTESIAN_POINT ( 'NONE',  ( -95.90974742083152194, -294.2893140455722119, -319.1279444767243376 ) ) ;
#41334=CARTESIAN_POINT ( 'NONE',  ( -81.97676093716518153, -296.9328507611767236, -212.4549782014388200 ) ) ;
#41336=CARTESIAN_POINT ( 'NONE',  ( -64.05433036862241636, -290.9270105524314545, -339.0972726322552262 ) ) ;
#41337=CARTESIAN_POINT ( 'NONE',  ( 36.52989528231221783, -283.2527311973069573, -265.7827555074986776 ) ) ;
#41339=CARTESIAN_POINT ( 'NONE',  ( -110.2143621876788302, -291.6844106967669177, -293.5160393329211388 ) ) ;
#41340=CARTESIAN_POINT ( 'NONE',  ( -70.41065345981498069, -290.7940611967126188, -339.3663976293753990 ) ) ;
#41341=CARTESIAN_POINT ( 'NONE',  ( -41.45747046174550121, -288.0005051087389916, -195.4612886322359202 ) ) ;
#41342=CARTESIAN_POINT ( 'NONE',  ( -11.51135464438669409, -280.5460374620005837, -197.7669172733149026 ) ) ;
#41343=CARTESIAN_POINT ( 'NONE',  ( -78.70941993553368832, -293.6846139679248608, -333.5910630584564274 ) ) ;
#41344=CARTESIAN_POINT ( 'NONE',  ( -38.73467545788268040, -282.9024924014703970, -347.3485171090485437 ) ) ;
#41346=CARTESIAN_POINT ( 'NONE',  ( 34.44256959712029698, -277.6582121440334845, -289.2789429787712265 ) ) ;
#41347=CARTESIAN_POINT ( 'NONE',  ( -67.74223827176244583, -282.1233781216987495, -207.3071070584150277 ) ) ;
#41348=CARTESIAN_POINT ( 'NONE',  ( 35.08984844880483678, -274.0845875652014456, -293.3316378803804696 ) ) ;
#41350=CARTESIAN_POINT ( 'NONE',  ( 34.62879086799097195, -280.8940019097055938, -257.7818943358235515 ) ) ;
#41352=CARTESIAN_POINT ( 'NONE',  ( -94.90223437500507941, -279.0696455736311350, -320.9060842645401976 ) ) ;
#41353=CARTESIAN_POINT ( 'NONE',  ( -10.06631755336795564, -285.4583106441060636, -198.5488340660893982 ) ) ;
#41354=CARTESIAN_POINT ( 'NONE',  ( 11.58409444775172936, -294.5017767363566463, -214.7568083912356087 ) ) ;
#41355=CARTESIAN_POINT ( 'NONE',  ( -63.30387613299685512, -275.3195813716937437, -198.7203067652910704 ) ) ;
#41356=CARTESIAN_POINT ( 'NONE',  ( -110.5700346080669760, -274.1492930871249314, -248.0234173299515419 ) ) ;
#41358=CARTESIAN_POINT ( 'NONE',  ( 34.70680804688093701, -275.5444737867629783, -282.4143692279272386 ) ) ;
#41359=CARTESIAN_POINT ( 'NONE',  ( -53.52155392867422279, -297.2602238345237993, -343.4776699596290541 ) ) ;
#41360=CARTESIAN_POINT ( 'NONE',  ( -22.06119998568924245, -284.2480557287098009, -197.0512943070299912 ) ) ;
#41361=CARTESIAN_POINT ( 'NONE',  ( -33.53616458209059914, -291.7655474367319925, -193.4763848375828843 ) ) ;
#41362=CARTESIAN_POINT ( 'NONE',  ( 36.25144443124563765, -273.4101979276783823, -257.7992226760327981 ) ) ;
#41363=CARTESIAN_POINT ( 'NONE',  ( 33.30834032176397130, -289.5201148833864409, -299.0501748027612052 ) ) ;
#41364=CARTESIAN_POINT ( 'NONE',  ( -103.8309236640189397, -289.8875277130449604, -239.4837925441728714 ) ) ;
#41366=CARTESIAN_POINT ( 'NONE',  ( 18.99360916416825518, -291.4191886706000787, -218.7380686725811074 ) ) ;
#41367=CARTESIAN_POINT ( 'NONE',  ( -94.30473399079460251, -290.8645809552307355, -224.6542686835606730 ) ) ;
#41369=CARTESIAN_POINT ( 'NONE',  ( 33.56834547272224967, -288.2575454174322545, -241.0118656208562129 ) ) ;
#41370=CARTESIAN_POINT ( 'NONE',  ( -108.1915638814336802, -278.6516486110755864, -288.0870483253908674 ) ) ;
#41371=CARTESIAN_POINT ( 'NONE',  ( 22.03853054096587627, -293.1268058947201780, -318.9150237479514090 ) ) ;
#41372=CARTESIAN_POINT ( 'NONE',  ( -114.0508273546338103, -285.2799104626408848, -264.2645916975442333 ) ) ;
#41373=CARTESIAN_POINT ( 'NONE',  ( -109.2816787757773227, -284.5369166733178758, -297.9027642643281979 ) ) ;
#41374=CARTESIAN_POINT ( 'NONE',  ( 35.58725195009324693, -281.9338106551800820, -274.0292831194072392 ) ) ;
#41375=CARTESIAN_POINT ( 'NONE',  ( 5.511235791697614239, -58.25811859054644515, -354.7422047037252355 ) ) ;
#41376=CARTESIAN_POINT ( 'NONE',  ( -72.21123258206935702, -195.3303827311551402, -359.1388006984578283 ) ) ;
#41377=CARTESIAN_POINT ( 'NONE',  ( 197.7106711174764655, 286.7663448939923114, -96.38273171682746465 ) ) ;
#41378=CARTESIAN_POINT ( 'NONE',  ( 25.50907715839022671, -275.2630468307652336, -307.8095027429330912 ) ) ;
#41379=CARTESIAN_POINT ( 'NONE',  ( -32.41345497286733490, -275.9090238474583998, -343.5545697824167632 ) ) ;
#41380=CARTESIAN_POINT ( 'NONE',  ( -101.4949129165882198, -296.6192087254643184, -227.8648787276140126 ) ) ;
#41381=CARTESIAN_POINT ( 'NONE',  ( -104.7359985975682974, -260.9361277188981489, -315.7277192616979846 ) ) ;
#41383=CARTESIAN_POINT ( 'NONE',  ( 22.24629620678343045, -274.8844703966639713, -318.3669252183344156 ) ) ;
#41384=CARTESIAN_POINT ( 'NONE',  ( -46.32367503924465524, -275.6967808600020930, -196.8948118342178759 ) ) ;
#41386=CARTESIAN_POINT ( 'NONE',  ( -109.6333203565924919, -297.8203368701824161, -244.5397729879170754 ) ) ;
#41387=CARTESIAN_POINT ( 'NONE',  ( 3.654318923425740273, -288.9766697818042189, -330.8978636715258403 ) ) ;
#41388=CARTESIAN_POINT ( 'NONE',  ( -108.2221221050199631, -296.9753003042635555, -300.1656769617289910 ) ) ;
#41389=CARTESIAN_POINT ( 'NONE',  ( -66.89500004176926495, -295.9215229857758800, -341.4114208345997099 ) ) ;
#41390=CARTESIAN_POINT ( 'NONE',  ( 28.39547615711503425, -294.1498093294815703, -302.2207882684590459 ) ) ;
#41392=CARTESIAN_POINT ( 'NONE',  ( 25.71512263424697409, -276.9143873373876659, -228.7299841902427318 ) ) ;
#41394=CARTESIAN_POINT ( 'NONE',  ( -31.07251517508866101, -279.6368727734683830, -193.6258493168994335 ) ) ;
#41396=CARTESIAN_POINT ( 'NONE',  ( -45.92381204645155890, -278.1047561628644758, -343.1426139705459946 ) ) ;
#41397=CARTESIAN_POINT ( 'NONE',  ( 21.05749831130191296, -276.6496372410165350, -221.7451983856155664 ) ) ;
#41398=CARTESIAN_POINT ( 'NONE',  ( -94.90932168836425831, -275.9027043147746667, -319.0058896495945078 ) ) ;
#41399=CARTESIAN_POINT ( 'NONE',  ( -95.37504497151657290, -297.8282749759426338, -225.8882324612126524 ) ) ;
#41400=CARTESIAN_POINT ( 'NONE',  ( -110.6354344245422254, -295.2202618890138410, -263.2246067501200173 ) ) ;
#41402=CARTESIAN_POINT ( 'NONE',  ( -50.93492052454265462, -280.3752551515775622, -194.6329774909152377 ) ) ;
#41403=CARTESIAN_POINT ( 'NONE',  ( 23.98553936077475512, -276.2681252530847473, -310.0519248803364576 ) ) ;
#41405=CARTESIAN_POINT ( 'NONE',  ( 15.96764387764321569, -285.4737880948593443, -215.4847832503679399 ) ) ;
#41406=CARTESIAN_POINT ( 'NONE',  ( -32.09572632087548527, -300.1178316423048500, -195.1926590726061193 ) ) ;
#41407=CARTESIAN_POINT ( 'NONE',  ( 82.62739761238445624, -301.2431227241796137, -197.2117082864666600 ) ) ;
#41409=CARTESIAN_POINT ( 'NONE',  ( 30.63142610091495754, -287.1122188855687227, -297.5579312345154790 ) ) ;
#41410=AXIS2_PLACEMENT_3D ( 'NONE', #61892, #60964, #24491 ) ;
#41411=CARTESIAN_POINT ( 'NONE',  ( -70.16984558620852397, -277.8534006830432190, -204.0124247109837370 ) ) ;
#41412=CARTESIAN_POINT ( 'NONE',  ( -59.89711201537725316, -278.3289551617787652, -200.2600583664776934 ) ) ;
#41413=CARTESIAN_POINT ( 'NONE',  ( -105.4402984434636323, -282.2352360419093884, -300.4259662696737223 ) ) ;
#41414=CARTESIAN_POINT ( 'NONE',  ( -65.75662015852823572, -287.6807968292244482, -200.8978323062794971 ) ) ;
#41415=CARTESIAN_POINT ( 'NONE',  ( -95.93797296480778414, -280.3749618890283273, -226.1406204970063527 ) ) ;
#41417=CARTESIAN_POINT ( 'NONE',  ( -36.42897949586679829, -294.0637537311178562, -195.3539741908275573 ) ) ;
#41418=CIRCLE ( 'NONE', #73225, 3.491568894204821749 ) ;
#41419=CARTESIAN_POINT ( 'NONE',  ( -102.7451726378532868, -276.2802090978213982, -309.1471627736226537 ) ) ;
#41420=CARTESIAN_POINT ( 'NONE',  ( 29.25053169632317918, -276.6094312538228337, -300.5168359889639191 ) ) ;
#41421=CARTESIAN_POINT ( 'NONE',  ( 36.18586380700367755, -283.3515133553473220, -254.6879192266613359 ) ) ;
#41422=DIRECTION ( 'NONE',  ( -1.000000000000000000, -0.000000000000000000, -0.000000000000000000 ) ) ;
#41423=CARTESIAN_POINT ( 'NONE',  ( -62.26515384258541985, -291.2938208454318669, -341.7476097961869641 ) ) ;
#41424=CARTESIAN_POINT ( 'NONE',  ( -87.43994764063363334, -293.7503938971767070, -326.2434960983061387 ) ) ;
#41425=CARTESIAN_POINT ( 'NONE',  ( -113.9899638730542932, -283.8258988624224912, -264.2508779054703609 ) ) ;
#41427=CARTESIAN_POINT ( 'NONE',  ( 13.85209836054729315, -273.4734954537382805, -217.6312547771131563 ) ) ;
#41428=CARTESIAN_POINT ( 'NONE',  ( -38.90015348860767830, -290.1719784934156223, -196.1422746456413222 ) ) ;
#41429=CARTESIAN_POINT ( 'NONE',  ( 202.9738562182569694, 296.4636489450776367, -53.99999999999997868 ) ) ;
#41431=CARTESIAN_POINT ( 'NONE',  ( -101.0939488831900519, -289.5893851261556620, -228.3335476889303379 ) ) ;
#41432=CARTESIAN_POINT ( 'NONE',  ( -101.0819459649954410, -285.6472829774787101, -307.5581806947480459 ) ) ;
#41433=CARTESIAN_POINT ( 'NONE',  ( 37.78711643400389164, -285.6466208005097656, -258.8885846512430930 ) ) ;
#41434=CARTESIAN_POINT ( 'NONE',  ( -102.7705054953186590, -286.4316196384670548, -236.6795749106795768 ) ) ;
#41435=CARTESIAN_POINT ( 'NONE',  ( -4.531289960885949597, -287.2988412736495434, -204.9693852317697917 ) ) ;
#41436=CARTESIAN_POINT ( 'NONE',  ( -78.71292160567136875, -293.4781675314818017, -207.3159641016412138 ) ) ;
#41437=CARTESIAN_POINT ( 'NONE',  ( 36.76519531547990738, -273.8199522145540072, -285.1083973468112163 ) ) ;
#41438=CARTESIAN_POINT ( 'NONE',  ( 39.60961237824037795, -275.8596739927569956, -268.3020417353718585 ) ) ;
#41439=CARTESIAN_POINT ( 'NONE',  ( -41.94140849047675346, -290.0744507505808656, -194.9412473780233768 ) ) ;
#41440=CARTESIAN_POINT ( 'NONE',  ( -110.6666676216834588, -278.2546883081078022, -294.0370261877187090 ) ) ;
#41441=CARTESIAN_POINT ( 'NONE',  ( -39.71666763639395015, -297.0619874879278655, -344.9808414646738015 ) ) ;
#41444=CARTESIAN_POINT ( 'NONE',  ( -105.6786303335850192, -282.8760221689911987, -297.5424248709305175 ) ) ;
#41445=CARTESIAN_POINT ( 'NONE',  ( -104.3762601446401703, -276.9975555546783994, -236.6097080058894448 ) ) ;
#41447=CARTESIAN_POINT ( 'NONE',  ( -31.29552210731097261, -272.6070602186015890, -194.2811993839129627 ) ) ;
#41448=CARTESIAN_POINT ( 'NONE',  ( -35.12284158092999320, -276.3721413132199700, -343.4293691948372498 ) ) ;
#41449=CARTESIAN_POINT ( 'NONE',  ( 33.79098080276330762, -295.3248334093859171, -289.6665972240092515 ) ) ;
#41450=CARTESIAN_POINT ( 'NONE',  ( 38.56335310471677502, -280.6099883000420618, -281.3117071650368644 ) ) ;
#41451=CARTESIAN_POINT ( 'NONE',  ( -73.40787444732877987, -296.4844850177152011, -334.0999563649610309 ) ) ;
#41452=CARTESIAN_POINT ( 'NONE',  ( -64.07806012873268742, -296.7089265687841930, -342.0442075254208021 ) ) ;
#41453=CARTESIAN_POINT ( 'NONE',  ( -36.48127492339978772, -297.8965383374562066, -197.3611431048962856 ) ) ;
#41454=CARTESIAN_POINT ( 'NONE',  ( -92.24004992895380894, -293.2675844134609520, -219.2424956665714433 ) ) ;
#41455=CARTESIAN_POINT ( 'NONE',  ( -112.3602088651110051, -284.9358911517914521, -253.0053307226875461 ) ) ;
#41456=CARTESIAN_POINT ( 'NONE',  ( 30.16071396225005330, -273.2414297244706631, -235.9557467476845716 ) ) ;
#41457=CARTESIAN_POINT ( 'NONE',  ( 31.68648011654244456, -287.8252788996738900, -304.6004228847726267 ) ) ;
#41458=CARTESIAN_POINT ( 'NONE',  ( -94.36262064907354841, -281.2016807607589612, -222.1702798802900531 ) ) ;
#41459=CARTESIAN_POINT ( 'NONE',  ( -85.87313592555500463, -284.4193181181659043, -215.4471252058430082 ) ) ;
#41460=CARTESIAN_POINT ( 'NONE',  ( -36.37780040960624461, -290.0640810599271617, -195.3546134821183671 ) ) ;
#41461=CARTESIAN_POINT ( 'NONE',  ( -72.39245198575343920, -211.1690049852372226, -355.6323962662157783 ) ) ;
#41463=CARTESIAN_POINT ( 'NONE',  ( 11.17960546522221321, -286.2532224697061451, -215.6701459217152888 ) ) ;
#41465=CARTESIAN_POINT ( 'NONE',  ( -2.987354850028779207, -283.5506475113002125, -339.0241008027304588 ) ) ;
#41466=CARTESIAN_POINT ( 'NONE',  ( -109.6479822902343955, -289.2827295766998077, -296.2990371597725812 ) ) ;
#41467=CARTESIAN_POINT ( 'NONE',  ( -84.09235222965038759, -281.0221604726231703, -210.1211068474909212 ) ) ;
#41468=CARTESIAN_POINT ( 'NONE',  ( -95.54163159470810740, -280.5416025944564353, -220.6814874622443767 ) ) ;
#41469=CARTESIAN_POINT ( 'NONE',  ( 15.26085450888212947, -280.6539499138401084, -219.6729841377985508 ) ) ;
#41470=CARTESIAN_POINT ( 'NONE',  ( 1.630558087549926150, -276.5734098269544461, -206.2817629779650872 ) ) ;
#41471=CARTESIAN_POINT ( 'NONE',  ( 17.56154560499861716, -294.2940206919910793, -324.4243018859324934 ) ) ;
#41473=CARTESIAN_POINT ( 'NONE',  ( -109.3316657499150466, -288.8272000385535989, -250.6306427063725266 ) ) ;
#41474=CARTESIAN_POINT ( 'NONE',  ( -79.89635740851900891, -296.3814757464465401, -210.6675067955377756 ) ) ;
#41477=CARTESIAN_POINT ( 'NONE',  ( -13.03653723666044861, -284.6541846856612779, -340.7760969264413689 ) ) ;
#41478=CARTESIAN_POINT ( 'NONE',  ( -77.96502750404248161, -295.2811527920156323, -331.1003016930922058 ) ) ;
#41479=CARTESIAN_POINT ( 'NONE',  ( 8.654503940854340271, -293.7452787957932401, -208.9283932366735712 ) ) ;
#41481=CARTESIAN_POINT ( 'NONE',  ( -33.48255945011700163, -283.6537431950467862, -343.3737060117775854 ) ) ;
#41483=CARTESIAN_POINT ( 'NONE',  ( -2.653111489142776502, -273.5582507639357459, -201.8663742341396699 ) ) ;
#41484=CARTESIAN_POINT ( 'NONE',  ( -111.5366392243365823, -291.4575787174883317, -250.1016344997444776 ) ) ;
#41485=CARTESIAN_POINT ( 'NONE',  ( -70.50386244415177828, -283.7591896734205079, -202.2393411752990744 ) ) ;
#41486=CARTESIAN_POINT ( 'NONE',  ( -91.58061881280454486, -290.1321316693956760, -325.0610376856986363 ) ) ;
#41487=CARTESIAN_POINT ( 'NONE',  ( 34.58747631600389383, -287.7157585265050557, -257.4950100333157366 ) ) ;
#41490=CARTESIAN_POINT ( 'NONE',  ( 193.0906159184471846, 275.7967025259000593, -123.9984796719191422 ) ) ;
#41491=CARTESIAN_POINT ( 'NONE',  ( -89.94602559131035946, -285.2986515701680332, -325.7100612913062037 ) ) ;
#41492=CARTESIAN_POINT ( 'NONE',  ( 21.27581636871891391, -285.6952119285919025, -317.1477375740089997 ) ) ;
#41494=CARTESIAN_POINT ( 'NONE',  ( 35.66151926106301318, -280.3775458185024263, -263.1344880193751123 ) ) ;
#41495=CARTESIAN_POINT ( 'NONE',  ( -4.007846544576714187, -276.2912354927674983, -339.7629202201153475 ) ) ;
#41496=CARTESIAN_POINT ( 'NONE',  ( -74.91222203738804808, -279.5539075092778489, -335.0796185089115511 ) ) ;
#41497=CARTESIAN_POINT ( 'NONE',  ( 175.6347583417331748, 240.9695037902932029, -178.4445647501395058 ) ) ;
#41499=CARTESIAN_POINT ( 'NONE',  ( 37.56430762138740675, -280.3170572111532692, -285.4507269113763073 ) ) ;
#41500=CARTESIAN_POINT ( 'NONE',  ( -94.49866316113217124, -283.2390678192696782, -222.3514483033902138 ) ) ;
#41501=CARTESIAN_POINT ( 'NONE',  ( -111.3141019553943210, -298.0913164673240203, -287.7971380697699715 ) ) ;
#41503=CARTESIAN_POINT ( 'NONE',  ( 25.84902749512648867, -294.5472004113508433, -307.0342741595256939 ) ) ;
#41505=CARTESIAN_POINT ( 'NONE',  ( -108.2231117701188339, -289.4918107992207865, -250.9428543479009761 ) ) ;
#41506=CARTESIAN_POINT ( 'NONE',  ( -39.95117398810393894, -277.7355083739330439, -347.2279465269218690 ) ) ;
#41507=CARTESIAN_POINT ( 'NONE',  ( -66.82128638378274843, -297.8214885693381575, -203.5645509084472167 ) ) ;
#41509=CARTESIAN_POINT ( 'NONE',  ( -24.19900087458676552, -273.1363941837475977, -194.7508178983115386 ) ) ;
#41514=CARTESIAN_POINT ( 'NONE',  ( 29.60232393066930001, -283.0339455442720578, -300.3642940624312700 ) ) ;
#41515=CARTESIAN_POINT ( 'NONE',  ( -4.580158049601985581, -284.3866045963768556, -338.9367445439181665 ) ) ;
#41516=CARTESIAN_POINT ( 'NONE',  ( -53.75402061754415683, -282.3265910824628122, -341.7859453671997585 ) ) ;
#41517=CARTESIAN_POINT ( 'NONE',  ( 36.25419105348277782, -283.2815160131809762, -260.2582051990389118 ) ) ;
#41518=CARTESIAN_POINT ( 'NONE',  ( 3.502449031520246336, -274.9716349172953755, -331.7000389930661868 ) ) ;
#41521=CARTESIAN_POINT ( 'NONE',  ( -41.36574395494807987, -277.9044063292082001, -347.1073812851673779 ) ) ;
#41525=CARTESIAN_POINT ( 'NONE',  ( -110.2955976910047582, -286.1521804467080869, -290.8070054030278584 ) ) ;
#41526=CARTESIAN_POINT ( 'NONE',  ( 23.06053835761465720, -293.3235401869716270, -311.7313027195789346 ) ) ;
#41527=CARTESIAN_POINT ( 'NONE',  ( 33.94471415763714361, -287.2689357643765788, -299.3396933785547276 ) ) ;
#41528=CARTESIAN_POINT ( 'NONE',  ( -24.95040502862489262, -284.4520589960428083, -197.3404152852579898 ) ) ;
#41529=CARTESIAN_POINT ( 'NONE',  ( -102.2998172363050458, -282.6581329209695355, -305.0502218231461597 ) ) ;
#41530=CARTESIAN_POINT ( 'NONE',  ( -99.70753367729410854, -288.2482962413515111, -310.2168179338679010 ) ) ;
#41531=CARTESIAN_POINT ( 'NONE',  ( -110.7066776044088243, -285.7857108612488446, -268.1907300975811381 ) ) ;
#41532=CARTESIAN_POINT ( 'NONE',  ( 7.036594990000758720, -274.4481728403393390, -330.8866921735930759 ) ) ;
#41533=CARTESIAN_POINT ( 'NONE',  ( -5.093791064963393289, -284.8694863026918824, -201.3211818632843233 ) ) ;
#41534=CARTESIAN_POINT ( 'NONE',  ( -15.56249213115096097, -300.3249431746697269, -195.3536842308016617 ) ) ;
#41535=CARTESIAN_POINT ( 'NONE',  ( -54.52028126809830866, -283.8317529060831816, -197.1837664763651219 ) ) ;
#41536=CARTESIAN_POINT ( 'NONE',  ( 35.58547329939473514, -282.3981436429428413, -263.1161870991642786 ) ) ;
#41538=CARTESIAN_POINT ( 'NONE',  ( 36.22384026247603828, -289.3538093336782140, -254.8671198385670209 ) ) ;
#41540=DIRECTION ( 'NONE',  ( 0.000000000000000000, 0.000000000000000000, -1.000000000000000000 ) ) ;
#41541=CARTESIAN_POINT ( 'NONE',  ( -92.61901793798266169, -297.7564623106414388, -321.8945566341897120 ) ) ;
#41542=CARTESIAN_POINT ( 'NONE',  ( -3.420831710505241929, -278.4997593246368410, -203.4560727217182148 ) ) ;
#41543=CARTESIAN_POINT ( 'NONE',  ( -112.4799072212602340, -289.9515286357162154, -254.2239865104348837 ) ) ;
#41544=CARTESIAN_POINT ( 'NONE',  ( -39.73517681792971246, -293.4825457400801270, -344.1348644714923921 ) ) ;
#41545=CARTESIAN_POINT ( 'NONE',  ( -101.2323203910118963, -277.7311004750494021, -234.0398828799493742 ) ) ;
#41546=CARTESIAN_POINT ( 'NONE',  ( -37.80687756199515093, -296.1858490380373610, -196.1273716551077655 ) ) ;
#41547=CARTESIAN_POINT ( 'NONE',  ( 32.01095838245846892, -295.1905251591877573, -294.8333896647420147 ) ) ;
#41548=CARTESIAN_POINT ( 'NONE',  ( -114.2704648735229114, -293.0519495502702512, -270.3937649182068981 ) ) ;
#41549=CARTESIAN_POINT ( 'NONE',  ( -113.5426982570904499, -294.9700149871536041, -275.2752556983063528 ) ) ;
#41550=CARTESIAN_POINT ( 'NONE',  ( -10.41340708330305453, -290.2951021242247407, -339.1277056067564217 ) ) ;
#41551=CARTESIAN_POINT ( 'NONE',  ( 21.43981081841886649, -291.1368129287019997, -222.2081535054409756 ) ) ;
#41553=CARTESIAN_POINT ( 'NONE',  ( -110.7085486079273551, -291.8944991757177263, -276.6985717526271742 ) ) ;
#41555=CARTESIAN_POINT ( 'NONE',  ( -83.93973002601904909, -292.1954752220521527, -213.9587657616031890 ) ) ;
#41557=CARTESIAN_POINT ( 'NONE',  ( -94.42570921331406453, -292.4536984853795047, -219.2785903849262468 ) ) ;
#41558=CARTESIAN_POINT ( 'NONE',  ( 18.91786417711920976, -278.8776249305042825, -220.2092013673012616 ) ) ;
#41559=CARTESIAN_POINT ( 'NONE',  ( 34.71394299542819795, -293.3967254417360095, -258.5789227502350514 ) ) ;
#41560=CARTESIAN_POINT ( 'NONE',  ( 37.67749848607583374, -281.3344768217687601, -252.9503824223577908 ) ) ;
#41561=CARTESIAN_POINT ( 'NONE',  ( -114.1304238725785893, -284.2953746480517907, -264.2456914075312966 ) ) ;
#41563=CARTESIAN_POINT ( 'NONE',  ( -67.08045649038925262, -287.4425783561480898, -339.0869808148911488 ) ) ;
#41564=CARTESIAN_POINT ( 'NONE',  ( -109.6335024211604008, -282.4721776528767236, -287.2915931714493922 ) ) ;
#41566=CARTESIAN_POINT ( 'NONE',  ( 20.55282127485811827, -279.3548368245381539, -220.6327715716640512 ) ) ;
#41568=CARTESIAN_POINT ( 'NONE',  ( -67.05654831457397336, -284.5919779865603800, -199.6609036442864067 ) ) ;
#41570=CARTESIAN_POINT ( 'NONE',  ( 36.33191401159005096, -295.0854739651622367, -265.2407560999006932 ) ) ;
#41571=CARTESIAN_POINT ( 'NONE',  ( 6.879091576360326421, -276.0658375190361085, -207.9814464762356181 ) ) ;
#41572=CARTESIAN_POINT ( 'NONE',  ( -108.1936299300499940, -277.9851940958232603, -288.0787889379510034 ) ) ;
#41573=CARTESIAN_POINT ( 'NONE',  ( -69.62509661333739075, -291.8055178983028668, -200.4412521545260688 ) ) ;
#41574=CARTESIAN_POINT ( 'NONE',  ( -92.39934421272458565, -281.9121035074234101, -322.1291997727531680 ) ) ;
#41576=CARTESIAN_POINT ( 'NONE',  ( 34.44951332011830658, -292.4206051034574330, -255.8894173084161423 ) ) ;
#41577=CARTESIAN_POINT ( 'NONE',  ( -94.08546788035883424, -293.8718696552895722, -319.4034004788132393 ) ) ;
#41580=CARTESIAN_POINT ( 'NONE',  ( -79.56115982651462559, -290.9724038011422067, -210.6710488745503369 ) ) ;
#41582=CARTESIAN_POINT ( 'NONE',  ( -21.39648532958014826, -274.3380690714489560, -340.3683826091709079 ) ) ;
#41583=CARTESIAN_POINT ( 'NONE',  ( -102.9208208713124293, -295.0882822397881000, -310.2634880261027206 ) ) ;
#41584=CARTESIAN_POINT ( 'NONE',  ( -7.993226794930098578, -278.5721042578804258, -200.4973993423118372 ) ) ;
#41585=CARTESIAN_POINT ( 'NONE',  ( -108.5754930492163766, -286.2250307942047698, -242.3055826994246615 ) ) ;
#41586=CARTESIAN_POINT ( 'NONE',  ( -19.81380064240008920, -286.1171645995170252, -199.4966505528033736 ) ) ;
#41587=CARTESIAN_POINT ( 'NONE',  ( 29.79379416280975335, -277.4780001990760638, -300.7508063137664749 ) ) ;
#41588=CARTESIAN_POINT ( 'NONE',  ( -87.61596725676020014, -293.7783860190706946, -325.5367001267342744 ) ) ;
#41589=CARTESIAN_POINT ( 'NONE',  ( -78.49482072034837188, -297.3742380632951949, -331.9404433679606541 ) ) ;
#41590=CARTESIAN_POINT ( 'NONE',  ( -109.8868493745971477, -277.2007750650690809, -281.5115361781025740 ) ) ;
#41593=CARTESIAN_POINT ( 'NONE',  ( -99.99376879883324420, -295.6252415433453393, -315.1774376555846970 ) ) ;
#41594=CARTESIAN_POINT ( 'NONE',  ( -66.87833645481680378, -291.3622593980742295, -338.7455489394475876 ) ) ;
#41596=CARTESIAN_POINT ( 'NONE',  ( -50.76204978943955126, -289.8794172020000701, -342.2723619224744880 ) ) ;
#41599=CARTESIAN_POINT ( 'NONE',  ( -50.88630447160315384, -278.9418867547200307, -194.8007850987532379 ) ) ;
#41600=CARTESIAN_POINT ( 'NONE',  ( -110.2464297723367821, -296.8951612652207359, -294.8195149453471231 ) ) ;
#41601=CARTESIAN_POINT ( 'NONE',  ( -102.1468385063062527, -289.2135586312229520, -231.0095459031336418 ) ) ;
#41602=CARTESIAN_POINT ( 'NONE',  ( -82.96146110630758130, -297.7805255820161960, -208.2901946683190317 ) ) ;
#41603=CARTESIAN_POINT ( 'NONE',  ( 21.81934756833250333, -293.2865567852622348, -227.5373111288986365 ) ) ;
#41607=CARTESIAN_POINT ( 'NONE',  ( -20.62923130197297539, -290.3615992699166668, -344.8693166486516475 ) ) ;
#41608=CARTESIAN_POINT ( 'NONE',  ( 13.84574458161073096, -278.9090924074131408, -334.4957818155094174 ) ) ;
#41610=CARTESIAN_POINT ( 'NONE',  ( 3.774488552245651718, -279.9382868265000752, -205.3153579709764358 ) ) ;
#41611=CARTESIAN_POINT ( 'NONE',  ( -108.2781457802385745, -286.8630330687701644, -246.3649136130257773 ) ) ;
#41612=CARTESIAN_POINT ( 'NONE',  ( 11.71330621739024913, -285.2922024623816242, -211.7069721845812182 ) ) ;
#41613=CARTESIAN_POINT ( 'NONE',  ( -90.52770824079732392, -271.2964016181175566, -217.7181985470718075 ) ) ;
#41614=CARTESIAN_POINT ( 'NONE',  ( -35.37634163115831853, -275.9971320135749693, -195.9343108153315711 ) ) ;
#41615=CARTESIAN_POINT ( 'NONE',  ( -110.0748593996025591, -288.4262529255840377, -286.2698117605277162 ) ) ;
#41616=CARTESIAN_POINT ( 'NONE',  ( 0.4517791500610099931, -278.4149966243742824, -336.0861389971571498 ) ) ;
#41618=CARTESIAN_POINT ( 'NONE',  ( -103.3698487317648187, -278.9742419918925407, -239.1089849171963237 ) ) ;
#41619=CARTESIAN_POINT ( 'NONE',  ( 35.45467088625077423, -280.8057350154866185, -263.1495266674969571 ) ) ;
#41620=CARTESIAN_POINT ( 'NONE',  ( -20.18183872319299610, -277.9164709957369723, -345.1620687583575204 ) ) ;
#41621=CARTESIAN_POINT ( 'NONE',  ( -113.3740930089107195, -277.2244783269777031, -280.1136452566762500 ) ) ;
#41622=CARTESIAN_POINT ( 'NONE',  ( 201.0614859237756775, 294.6279256560665090, -68.41024071426262765 ) ) ;
#41623=CARTESIAN_POINT ( 'NONE',  ( -13.14803923713535561, -275.3002158549089131, -197.5086164110182096 ) ) ;
#41625=CARTESIAN_POINT ( 'NONE',  ( -35.50789907027257186, -299.4999520329629945, -193.9499080600656669 ) ) ;
#41626=CARTESIAN_POINT ( 'NONE',  ( 21.27581636871892101, -289.4090924074130839, -223.5744983911110353 ) ) ;
#41628=CARTESIAN_POINT ( 'NONE',  ( 82.63923273776656231, -300.3135941503064714, -192.9728626493033801 ) ) ;
#41629=CARTESIAN_POINT ( 'NONE',  ( 23.78423427710064431, -288.0715849740251997, -229.7989241006791303 ) ) ;
#41630=CARTESIAN_POINT ( 'NONE',  ( 25.50647157808987231, -288.7413759433204063, -227.6286188763099005 ) ) ;
#41632=CARTESIAN_POINT ( 'NONE',  ( 23.58988187244508694, -287.4606736498562327, -310.7725284359871125 ) ) ;
#41633=CARTESIAN_POINT ( 'NONE',  ( -106.6209770983899148, -284.4895264130075248, -236.8960812199129293 ) ) ;
#41634=CARTESIAN_POINT ( 'NONE',  ( -8.920632395264135539, -278.8301062886173440, -202.2532379311441844 ) ) ;
#41635=CARTESIAN_POINT ( 'NONE',  ( -84.44968318218414538, -287.2565238148146136, -212.9209421357792849 ) ) ;
#41636=CARTESIAN_POINT ( 'NONE',  ( 33.78783447648743277, -279.7793127673329536, -251.0437210441863272 ) ) ;
#41637=CARTESIAN_POINT ( 'NONE',  ( -109.3739208729831347, -280.0592136932062317, -255.7169522442660536 ) ) ;
#41638=CARTESIAN_POINT ( 'NONE',  ( -51.28649568409007031, -277.7276336572794548, -342.0795334584285570 ) ) ;
#41639=CARTESIAN_POINT ( 'NONE',  ( 12.14755339502901421, -287.1761069587424799, -328.8318157996811237 ) ) ;
#41641=CARTESIAN_POINT ( 'NONE',  ( 11.39808363886833398, -283.1992571258298881, -329.8319329765034809 ) ) ;
#41642=CARTESIAN_POINT ( 'NONE',  ( -96.21917046797801731, -284.3768480404935417, -319.9089714645272693 ) ) ;
#41643=CARTESIAN_POINT ( 'NONE',  ( 34.06475212451169199, -281.5179630639535162, -255.1319065323168900 ) ) ;
#41647=CARTESIAN_POINT ( 'NONE',  ( -103.5423949123394749, -292.8980245138036480, -233.5131399065905669 ) ) ;
#41648=CARTESIAN_POINT ( 'NONE',  ( 3.889958749570145091, -291.2793407527752834, -205.8526114901084156 ) ) ;
#41649=CARTESIAN_POINT ( 'NONE',  ( 34.60689690629411075, -274.4311759228303913, -256.6933517624825640 ) ) ;
#41650=CARTESIAN_POINT ( 'NONE',  ( 1.710513562695761713, -293.8927571321402752, -336.6048904627697311 ) ) ;
#41651=CARTESIAN_POINT ( 'NONE',  ( -71.51127199249741295, -287.9918936810018977, -335.6681638812212896 ) ) ;
#41652=CARTESIAN_POINT ( 'NONE',  ( 2.808777516213296632, -290.8384062685925642, -208.1239280299051586 ) ) ;
#41653=CARTESIAN_POINT ( 'NONE',  ( -94.40335296259695497, -291.1077805326222006, -316.5249380365361276 ) ) ;
#41655=CARTESIAN_POINT ( 'NONE',  ( -112.3885822208017515, -292.5411397846005457, -271.2316422452453821 ) ) ;
#41656=CARTESIAN_POINT ( 'NONE',  ( -39.14163571056497659, -290.0294877915744678, -195.2032754166945949 ) ) ;
#41657=CARTESIAN_POINT ( 'NONE',  ( 8.939620280993420209, -294.6867878811980290, -211.2785924188806064 ) ) ;
#41658=CARTESIAN_POINT ( 'NONE',  ( -6.929696902326653252, -287.4025858886413971, -203.7251408791647975 ) ) ;
#41659=CARTESIAN_POINT ( 'NONE',  ( 37.41658326311324601, -295.6587166311339843, -278.6663784264282526 ) ) ;
#41661=CARTESIAN_POINT ( 'NONE',  ( 37.91014550762238855, -277.4701774622000130, -265.5197760581237958 ) ) ;
#41662=CARTESIAN_POINT ( 'NONE',  ( -103.7051730876373767, -296.2555370279769136, -231.5258277155712392 ) ) ;
#41663=CARTESIAN_POINT ( 'NONE',  ( -40.57212219243000106, -275.3331529661656418, -344.3165599633954344 ) ) ;
#41664=CARTESIAN_POINT ( 'NONE',  ( -111.0440694423989214, -276.7718420363114546, -259.5508040766388831 ) ) ;
#41665=CARTESIAN_POINT ( 'NONE',  ( -103.5699316611706706, -274.1827799328040669, -238.7232948651893878 ) ) ;
#41666=CARTESIAN_POINT ( 'NONE',  ( -84.84472907284245480, -297.1471853337678795, -326.6315422115357592 ) ) ;
#41668=CARTESIAN_POINT ( 'NONE',  ( -108.4535525103710398, -297.1279464807188901, -287.6100276268018092 ) ) ;
#41670=CARTESIAN_POINT ( 'NONE',  ( 37.99618899985917864, -285.5516144945797237, -268.7457971012664188 ) ) ;
#41671=CARTESIAN_POINT ( 'NONE',  ( -66.81933986555078775, -297.6548354787283870, -203.5636919474551689 ) ) ;
#41672=CARTESIAN_POINT ( 'NONE',  ( 7.543931294060559622, -286.6455329396953289, -207.7312399161872349 ) ) ;
#41673=CARTESIAN_POINT ( 'NONE',  ( -98.14551663014650273, -289.5882481465149567, -317.5695938150835786 ) ) ;
#41674=CARTESIAN_POINT ( 'NONE',  ( -82.01617823731210422, -299.4268715949281159, -209.6118577671483365 ) ) ;
#41675=CARTESIAN_POINT ( 'NONE',  ( 17.48543136529931274, -292.2661600562431659, -321.2925825132865043 ) ) ;
#41676=CARTESIAN_POINT ( 'NONE',  ( 23.62543954828221260, -280.1239585154711449, -223.5724660165973603 ) ) ;
#41677=CARTESIAN_POINT ( 'NONE',  ( -37.30987171927208834, -295.5523547857347353, -195.3611179825600175 ) ) ;
#41679=CARTESIAN_POINT ( 'NONE',  ( -73.75522210830541781, -288.3420212531743800, -334.1030439030342905 ) ) ;
#41681=CARTESIAN_POINT ( 'NONE',  ( -79.31421646316049134, -287.6181027514745097, -332.5791718530181242 ) ) ;
#41682=CARTESIAN_POINT ( 'NONE',  ( -105.0240918310044407, -274.4618434606221626, -241.0803634061171294 ) ) ;
#41683=CARTESIAN_POINT ( 'NONE',  ( 20.60729127639539016, -282.2997550093975292, -220.5364024447617339 ) ) ;
#41684=CARTESIAN_POINT ( 'NONE',  ( -83.20455907463373535, -293.6964141724263300, -330.2182697912767253 ) ) ;
#41685=CARTESIAN_POINT ( 'NONE',  ( 33.94041483488990707, -281.7598360453405917, -286.1046908428020288 ) ) ;
#41686=CARTESIAN_POINT ( 'NONE',  ( -77.08040976879073014, -295.7354882012526218, -336.3764263417740494 ) ) ;
#41687=CARTESIAN_POINT ( 'NONE',  ( 95.96543556739594294, -301.2707763474030571, -196.6326178096987860 ) ) ;
#41689=CARTESIAN_POINT ( 'NONE',  ( 36.46215972292451113, -283.7245304312448866, -283.7739075632489971 ) ) ;
#41690=CARTESIAN_POINT ( 'NONE',  ( -41.87095832627058201, -297.0524230194331494, -197.2660137102401734 ) ) ;
#41693=CARTESIAN_POINT ( 'NONE',  ( -112.0361296218977145, -286.5244943658366310, -270.9468144176681221 ) ) ;
#41695=CARTESIAN_POINT ( 'NONE',  ( 13.79469577742117181, -273.9094976428776818, -334.5364918783848793 ) ) ;
#41696=CARTESIAN_POINT ( 'NONE',  ( 31.70568146570080970, -275.1844804328716805, -304.1960407099032864 ) ) ;
#41697=CARTESIAN_POINT ( 'NONE',  ( -7.268306688921768455, -292.2912716140305065, -203.8435187205360251 ) ) ;
#41698=CARTESIAN_POINT ( 'NONE',  ( -59.13487383315286650, -284.8593530868857897, -340.8119567251113153 ) ) ;
#41700=CARTESIAN_POINT ( 'NONE',  ( 18.04901839466556979, -277.8412556586205824, -319.1480958424884307 ) ) ;
#41701=CARTESIAN_POINT ( 'NONE',  ( -111.6419001824270225, -285.7519484915279122, -288.2514335980770852 ) ) ;
#41702=CARTESIAN_POINT ( 'NONE',  ( -89.18557169189418232, -282.5961383796832251, -322.3876777027833782 ) ) ;
#41703=CARTESIAN_POINT ( 'NONE',  ( -70.65085845100729500, -281.6130930223119435, -203.1494154472848095 ) ) ;
#41704=CARTESIAN_POINT ( 'NONE',  ( 37.63442460701440240, -275.4988421891508779, -252.7657895295491528 ) ) ;
#41705=CARTESIAN_POINT ( 'NONE',  ( 23.51674089509399224, -276.0155820897891772, -317.5550585629911211 ) ) ;
#41706=CARTESIAN_POINT ( 'NONE',  ( -96.73884558491587882, -297.8539093632993513, -315.2518449888248711 ) ) ;
#41710=CARTESIAN_POINT ( 'NONE',  ( -102.0727733461083346, -294.1692663981784222, -309.7336164939565037 ) ) ;
#41711=CARTESIAN_POINT ( 'NONE',  ( 35.41472029519250242, -275.1477191736769896, -277.0313300294994860 ) ) ;
#41712=CARTESIAN_POINT ( 'NONE',  ( -60.31413826022249225, -287.5103150477829672, -200.0031681948654239 ) ) ;
#41713=CARTESIAN_POINT ( 'NONE',  ( -25.00069408847846830, -296.4177634806480341, -345.7168059011630703 ) ) ;
#41714=CARTESIAN_POINT ( 'NONE',  ( 19.24677467267338926, -295.4634734750544567, -322.0693317182562510 ) ) ;
#41715=CARTESIAN_POINT ( 'NONE',  ( -96.38164189535217474, -291.9200719071964727, -316.3634780867970449 ) ) ;
#41716=CARTESIAN_POINT ( 'NONE',  ( -108.0035765230149991, -276.2304972260376417, -295.1543290588861623 ) ) ;
#41717=CARTESIAN_POINT ( 'NONE',  ( -111.6030148488140981, -280.3965702138244751, -276.2160208940152870 ) ) ;
#41718=CARTESIAN_POINT ( 'NONE',  ( -106.3049748690865783, -294.2638691184287723, -298.3857666423747332 ) ) ;
#41719=CARTESIAN_POINT ( 'NONE',  ( -19.19097222564238336, -284.6815656523039593, -343.9737227675237818 ) ) ;
#41720=CARTESIAN_POINT ( 'NONE',  ( -96.00507022231452936, -284.0870177650495521, -226.3970976523370666 ) ) ;
#41721=CARTESIAN_POINT ( 'NONE',  ( 7.521071455173375497, -59.59353953422439076, -353.8445329526322780 ) ) ;
#41723=CARTESIAN_POINT ( 'NONE',  ( -105.2351610430884534, -283.8577569231067059, -297.3793561735712387 ) ) ;
#41725=CARTESIAN_POINT ( 'NONE',  ( 35.87648806123711864, -282.3440265301103977, -247.5446890760673000 ) ) ;
#41726=CARTESIAN_POINT ( 'NONE',  ( -103.6888315564941649, -283.8486317876976273, -231.9664155074464134 ) ) ;
#41727=CARTESIAN_POINT ( 'NONE',  ( -107.3565628231119859, -279.0887027739138944, -301.9664277389737777 ) ) ;
#41730=CARTESIAN_POINT ( 'NONE',  ( -9.447083545083982514, -278.2142350011095573, -341.3864523252224217 ) ) ;
#41731=CARTESIAN_POINT ( 'NONE',  ( 3.760469193432061097, -281.2409032959117212, -205.3064978043875044 ) ) ;
#41732=CARTESIAN_POINT ( 'NONE',  ( -53.35057174420112602, -300.3376638359844719, -200.3683826091709648 ) ) ;
#41733=CARTESIAN_POINT ( 'NONE',  ( 162.3984126888688877, 219.7162322416178597, -205.2442872645431748 ) ) ;
#41735=CARTESIAN_POINT ( 'NONE',  ( 23.76348346342304652, -276.9638032030176760, -227.1395828135516126 ) ) ;
#41736=CARTESIAN_POINT ( 'NONE',  ( -48.68011135779718046, -154.6331602903188696, -364.9585083841176925 ) ) ;
#41737=CARTESIAN_POINT ( 'NONE',  ( -69.20298245349890465, -277.6510244092736457, -202.8577440260321794 ) ) ;
#41738=CARTESIAN_POINT ( 'NONE',  ( 31.26132543115433293, -294.8864756245884564, -237.5647813649045759 ) ) ;
#41739=CARTESIAN_POINT ( 'NONE',  ( -6.729768481844214278, -293.9878953299498221, -336.7448683241781850 ) ) ;
#41740=CARTESIAN_POINT ( 'NONE',  ( -100.6335452153688124, -289.4816391902241435, -314.1066234512865094 ) ) ;
#41742=CARTESIAN_POINT ( 'NONE',  ( -58.70412568069531289, -293.8977481573832051, -343.7801090511866278 ) ) ;
#41743=CARTESIAN_POINT ( 'NONE',  ( -69.10094620801039866, -284.0271802005248105, -203.7304346851486514 ) ) ;
#41744=CARTESIAN_POINT ( 'NONE',  ( -44.44153510163963006, -293.8219487703494224, -196.4145287119885950 ) ) ;
#41745=CARTESIAN_POINT ( 'NONE',  ( -80.90507619547820184, -284.9723917196544107, -329.6145901829643208 ) ) ;
#41746=ORIENTED_EDGE ( 'NONE', *, *, #61930, .T. ) ;
#41747=CARTESIAN_POINT ( 'NONE',  ( -90.63125093652246278, -292.2606380785858846, -215.0329754065286068 ) ) ;
#41748=CARTESIAN_POINT ( 'NONE',  ( 20.23333590796336523, -282.6779471400249690, -315.3400426842292745 ) ) ;
#41749=CARTESIAN_POINT ( 'NONE',  ( -50.41493378120410540, -294.0102974119830037, -345.8939175681458096 ) ) ;
#41750=CARTESIAN_POINT ( 'NONE',  ( 10.13621599041971422, -289.2195304871756321, -330.8440964674711040 ) ) ;
#41752=CARTESIAN_POINT ( 'NONE',  ( -68.02357214386728401, -289.9366709306814300, -340.9171215045449799 ) ) ;
#41753=CARTESIAN_POINT ( 'NONE',  ( 22.75110663907214104, -288.2963254169742413, -311.8301617820586671 ) ) ;
#41756=CARTESIAN_POINT ( 'NONE',  ( -111.6814052290836230, -298.5993105178982887, -255.6685047828887605 ) ) ;
#41757=CARTESIAN_POINT ( 'NONE',  ( -57.24517541272127374, -296.4855112107333071, -196.4336717589160060 ) ) ;
#41759=CARTESIAN_POINT ( 'NONE',  ( 20.70976343061323277, -279.9843449149510093, -225.6928195841554157 ) ) ;
#41761=CARTESIAN_POINT ( 'NONE',  ( 19.30376808285199175, -298.0924932148090534, -193.4691040211189090 ) ) ;
#41762=CARTESIAN_POINT ( 'NONE',  ( -70.04903514772988160, -293.9710051964875106, -336.3985164054278130 ) ) ;
#41763=CARTESIAN_POINT ( 'NONE',  ( 35.71099084174209537, -277.4709839282748476, -282.5574158634472042 ) ) ;
#41764=CARTESIAN_POINT ( 'NONE',  ( -77.20793339934965616, -271.6510381350398120, -207.7388461943276923 ) ) ;
#41765=CARTESIAN_POINT ( 'NONE',  ( -20.74354049236241337, -296.0395239726513523, -341.9091842634544491 ) ) ;
#41766=CARTESIAN_POINT ( 'NONE',  ( -5.394424088937386230, -295.7013090630406964, -336.3567863077590800 ) ) ;
#41768=CARTESIAN_POINT ( 'NONE',  ( -69.17495047838239941, -297.0640410419794648, -339.6075056637247371 ) ) ;
#41769=CARTESIAN_POINT ( 'NONE',  ( -77.20801665719200457, -295.5188283460266234, -206.6374549372561376 ) ) ;
#41770=CARTESIAN_POINT ( 'NONE',  ( -86.00305685567641945, -292.0081559091677263, -215.7405716127899211 ) ) ;
#41771=CARTESIAN_POINT ( 'NONE',  ( -34.12021816225008308, -274.8945311294402813, -193.5901542346542215 ) ) ;
#41772=CARTESIAN_POINT ( 'NONE',  ( -108.6751992140893037, -289.3642052792698678, -252.2293552061949811 ) ) ;
#41774=CARTESIAN_POINT ( 'NONE',  ( -32.69259138734448555, -274.6015834248199212, -193.5501087911893023 ) ) ;
#41775=CARTESIAN_POINT ( 'NONE',  ( -100.1825056089172108, -296.3733661951385443, -307.6510001221028006 ) ) ;
#41776=CARTESIAN_POINT ( 'NONE',  ( 22.42698246003470430, -282.9062330948988802, -224.4476578473702659 ) ) ;
#41777=CARTESIAN_POINT ( 'NONE',  ( 3.572488707568652444, -279.2746329902387288, -205.6508138377376724 ) ) ;
#41778=CARTESIAN_POINT ( 'NONE',  ( -48.48742303607134119, -276.5389311568097241, -346.5009828279039539 ) ) ;
#41779=CARTESIAN_POINT ( 'NONE',  ( 37.07975229812336693, -280.1596354939910043, -286.7885837395131716 ) ) ;
#41780=CARTESIAN_POINT ( 'NONE',  ( 24.78017994419907311, -278.9792107219777790, -227.9512250103759641 ) ) ;
#41781=CARTESIAN_POINT ( 'NONE',  ( -76.86552517544035368, -272.0861116446538404, -208.2866290991796063 ) ) ;
#41782=CARTESIAN_POINT ( 'NONE',  ( -99.60396546988273769, -281.1180038728288650, -228.5242565469726799 ) ) ;
#41785=CARTESIAN_POINT ( 'NONE',  ( -62.48828682775742749, -295.9692418881478488, -198.6560052633979012 ) ) ;
#41786=CARTESIAN_POINT ( 'NONE',  ( 30.71162955993893462, -291.1470440113635618, -237.8800528281001334 ) ) ;
#41787=CARTESIAN_POINT ( 'NONE',  ( -74.67889708995357978, -291.5693216877177179, -203.0192014444159270 ) ) ;
#41788=CARTESIAN_POINT ( 'NONE',  ( 37.48952540902096331, -277.4546810752640909, -262.7402752453760968 ) ) ;
#41789=CARTESIAN_POINT ( 'NONE',  ( -3.171342694323064926, -272.5032799732290982, -203.5830308869954877 ) ) ;
#41791=CARTESIAN_POINT ( 'NONE',  ( 3.782857655889125592, -284.4238637016883331, -333.8113350966390840 ) ) ;
#41793=CARTESIAN_POINT ( 'NONE',  ( 34.12633415019790561, -285.8460164134294246, -293.1478109287773464 ) ) ;
#41795=CARTESIAN_POINT ( 'NONE',  ( -50.55768478198633886, -294.0196223028262921, -342.5585435140632740 ) ) ;
#41796=CARTESIAN_POINT ( 'NONE',  ( -6.481770789091785723, -284.6013712154704081, -202.8302678869715692 ) ) ;
#41798=CARTESIAN_POINT ( 'NONE',  ( -50.85592009661865376, -293.2246655496550147, -344.1335146128425322 ) ) ;
#41799=CARTESIAN_POINT ( 'NONE',  ( -94.82529980900078215, -282.3472038480871902, -320.5442179421402216 ) ) ;
#41800=CARTESIAN_POINT ( 'NONE',  ( -41.11221562341206948, -281.6040378283707923, -196.6574977922192886 ) ) ;
#41801=CARTESIAN_POINT ( 'NONE',  ( -1.170669037677460222, -287.7263251712611236, -202.8358247273881432 ) ) ;
#41802=CARTESIAN_POINT ( 'NONE',  ( 36.55755895016432078, -280.0168397491460723, -288.1047801723910879 ) ) ;
#41803=CARTESIAN_POINT ( 'NONE',  ( 30.97459740206149803, -287.2071295239269375, -244.4913271381309983 ) ) ;
#41804=CARTESIAN_POINT ( 'NONE',  ( -14.14017566206672605, -281.7842070762887943, -200.4712716021699066 ) ) ;
#41805=CARTESIAN_POINT ( 'NONE',  ( -27.54685636486275868, -280.9824608197324096, -197.8069680105778616 ) ) ;
#41806=CARTESIAN_POINT ( 'NONE',  ( 15.13529776561737528, -288.7683233690289626, -216.2818105420631980 ) ) ;
#41808=CARTESIAN_POINT ( 'NONE',  ( 53.58966561814242624, -298.9944938268030228, -193.3635553575743984 ) ) ;
#41809=CARTESIAN_POINT ( 'NONE',  ( -105.0588228997770557, -292.9465989243751665, -238.9566902197576042 ) ) ;
#41811=CARTESIAN_POINT ( 'NONE',  ( -37.37352853689063181, -300.5519495502701375, -190.3611179825600175 ) ) ;
#41812=ORIENTED_EDGE ( 'NONE', *, *, #5059, .F. ) ;
#41813=CARTESIAN_POINT ( 'NONE',  ( -2.137042854149974414, -272.5169823304725014, -203.9483139813929427 ) ) ;
#41814=CARTESIAN_POINT ( 'NONE',  ( -69.21208553357716653, -293.8643020225778741, -339.5904229530310658 ) ) ;
#41815=CARTESIAN_POINT ( 'NONE',  ( -71.68839007505155791, -297.0930535614419910, -205.8620784804440973 ) ) ;
#41816=CARTESIAN_POINT ( 'NONE',  ( 21.74085038285266336, -289.6846729316810070, -314.4272254184750182 ) ) ;
#41817=CARTESIAN_POINT ( 'NONE',  ( 14.02243007738041314, -282.5447841570524474, -217.0008812081251222 ) ) ;
#41818=CARTESIAN_POINT ( 'NONE',  ( -86.98771432678967130, -291.1524935598838510, -328.5157067783189291 ) ) ;
#41819=CARTESIAN_POINT ( 'NONE',  ( -67.84179295458659453, -290.7593647584248515, -340.5255150182598527 ) ) ;
#41820=CARTESIAN_POINT ( 'NONE',  ( -19.36036283374808420, -288.2836563955695510, -197.5485355892342056 ) ) ;
#41821=CARTESIAN_POINT ( 'NONE',  ( -98.57764851473837098, -279.3413593344394599, -223.6581797274827466 ) ) ;
#41822=CARTESIAN_POINT ( 'NONE',  ( 22.86645927910179665, -292.2518661865717036, -316.0151620746462413 ) ) ;
#41823=CARTESIAN_POINT ( 'NONE',  ( 20.13010064881657257, -280.6905442306977534, -219.0968566879743094 ) ) ;
#41824=CARTESIAN_POINT ( 'NONE',  ( 33.28044864426563265, -277.7110339564296737, -293.2385650201309772 ) ) ;
#41825=CARTESIAN_POINT ( 'NONE',  ( -92.08974858914540107, -281.6948066931272479, -226.7417163044926838 ) ) ;
#41826=CARTESIAN_POINT ( 'NONE',  ( 32.08471656633341951, -274.1914893272100926, -301.2471451849967252 ) ) ;
#41828=CARTESIAN_POINT ( 'NONE',  ( 33.17462298238724827, -280.8069214334814774, -251.1968409042158896 ) ) ;
#41829=CARTESIAN_POINT ( 'NONE',  ( -86.82692729869314974, -278.9275873386572471, -328.9046151632535384 ) ) ;
#41830=CARTESIAN_POINT ( 'NONE',  ( -66.02092967001290447, -274.9839746959575564, -202.6946915088247749 ) ) ;
#41831=CARTESIAN_POINT ( 'NONE',  ( -37.96846180250446423, -285.1032326207889014, -193.5989698632314173 ) ) ;
#41832=CARTESIAN_POINT ( 'NONE',  ( -101.1665947577201621, -291.8035560310515280, -307.9367605296737906 ) ) ;
#41833=CARTESIAN_POINT ( 'NONE',  ( -80.81091470282231626, -275.0735625324317652, -207.7122821438863980 ) ) ;
#41834=CARTESIAN_POINT ( 'NONE',  ( -100.8088841455731597, -274.4348457224380127, -227.5442398412263287 ) ) ;
#41835=CARTESIAN_POINT ( 'NONE',  ( 82.64890176555634582, -299.5541904835127980, -195.3611179825600175 ) ) ;
#41836=CARTESIAN_POINT ( 'NONE',  ( 5.395067839312406299, -276.2891231396670264, -329.6060420001832654 ) ) ;
#41837=CARTESIAN_POINT ( 'NONE',  ( -105.5986415013631472, -298.1477255315018624, -301.1637126802027637 ) ) ;
#41838=CARTESIAN_POINT ( 'NONE',  ( -80.34244608713942171, -283.4684023586116268, -209.0524005957549889 ) ) ;
#41839=CARTESIAN_POINT ( 'NONE',  ( 6.487675469906672099, -292.2968144910672663, -207.0781808972672309 ) ) ;
#41840=CARTESIAN_POINT ( 'NONE',  ( 35.77061901868826510, -273.7663918847093782, -285.4088950623718688 ) ) ;
#41841=CARTESIAN_POINT ( 'NONE',  ( 23.51571138032539210, -289.7692768306808375, -316.2175884309407365 ) ) ;
#41842=CARTESIAN_POINT ( 'NONE',  ( -109.5789663791787660, -289.6403510633914493, -257.5814579526740431 ) ) ;
#41844=CARTESIAN_POINT ( 'NONE',  ( -104.0864034529987094, -289.6128653067518712, -233.1623159914257144 ) ) ;
#41845=CARTESIAN_POINT ( 'NONE',  ( -109.4406586793314489, -290.0652698400853069, -282.0081835085784974 ) ) ;
#41846=VERTEX_POINT ( 'NONE', #89867 ) ;
#41847=CARTESIAN_POINT ( 'NONE',  ( 39.04081402945485735, -288.7180930021364702, -277.2316376238222233 ) ) ;
#41848=CARTESIAN_POINT ( 'NONE',  ( -107.6398201698862209, -279.1470379476784842, -250.5597196312261872 ) ) ;
#41849=CARTESIAN_POINT ( 'NONE',  ( -92.48433814451546198, -294.7394129464480557, -323.6601046720264208 ) ) ;
#41850=CARTESIAN_POINT ( 'NONE',  ( -105.6897389913451235, -284.7474459712592534, -305.7172865382960367 ) ) ;
#41851=CARTESIAN_POINT ( 'NONE',  ( -105.7634070545326068, -284.4293651346633283, -305.7508317293314235 ) ) ;
#41852=CARTESIAN_POINT ( 'NONE',  ( 21.02936191867633653, -282.5015535409899599, -314.2555394901853560 ) ) ;
#41853=CARTESIAN_POINT ( 'NONE',  ( -12.84209639897599331, -91.63111746082969944, -360.1199121724810652 ) ) ;
#41854=CARTESIAN_POINT ( 'NONE',  ( -40.89730568847058834, -138.9793244955967566, -363.4251286451764145 ) ) ;
#41855=CARTESIAN_POINT ( 'NONE',  ( 192.0717789903930282, 276.6821163107279631, -124.1503466236808606 ) ) ;
#41856=CARTESIAN_POINT ( 'NONE',  ( 29.23723054607156868, -274.3398496504575519, -239.9095363816517192 ) ) ;
#41857=CARTESIAN_POINT ( 'NONE',  ( 0.7849195434376035063, -273.4940745938593523, -207.7465274629228418 ) ) ;
#41858=CARTESIAN_POINT ( 'NONE',  ( -22.11586145835835282, -294.3697736302283943, -345.7779645081329818 ) ) ;
#41859=CARTESIAN_POINT ( 'NONE',  ( -110.4703370556568274, -271.6448334738088306, -283.7149836808490591 ) ) ;
#41860=CARTESIAN_POINT ( 'NONE',  ( 39.21375012171231589, -274.2473265192939493, -271.1831682273236765 ) ) ;
#41861=CARTESIAN_POINT ( 'NONE',  ( -110.9643546477779239, -298.5410764386292044, -260.4550081734931268 ) ) ;
#41862=CARTESIAN_POINT ( 'NONE',  ( -98.56523825880174172, -292.1897704973823124, -229.9463785342367430 ) ) ;
#41864=CARTESIAN_POINT ( 'NONE',  ( -112.3726326459767648, -297.2898888310659231, -286.5839222873647714 ) ) ;
#41865=CARTESIAN_POINT ( 'NONE',  ( 16.06022524577605992, -288.7617109895744534, -320.2971887779788176 ) ) ;
#41866=CARTESIAN_POINT ( 'NONE',  ( -99.87112668147683792, -296.7611718172383348, -315.1075192663511189 ) ) ;
#41867=CARTESIAN_POINT ( 'NONE',  ( -11.07232150900850698, -295.2112240252720881, -342.7325570573085542 ) ) ;
#41868=CARTESIAN_POINT ( 'NONE',  ( 27.15906500562259751, -294.1858136088330298, -304.6546838007758993 ) ) ;
#41870=CARTESIAN_POINT ( 'NONE',  ( 30.57194676240640518, -277.9070289200757884, -303.6021289741994451 ) ) ;
#41873=CARTESIAN_POINT ( 'NONE',  ( -38.16295524897140012, -279.5497740893025025, -193.4270394245857858 ) ) ;
#41874=CARTESIAN_POINT ( 'NONE',  ( 5.304060844957506404, -275.5860567421741507, -210.7606646313418821 ) ) ;
#41875=CARTESIAN_POINT ( 'NONE',  ( -8.101517869821336149, -276.1899073587616726, -200.1697926859102381 ) ) ;
#41876=CARTESIAN_POINT ( 'NONE',  ( -112.0823112359125133, -276.7000599708243840, -260.3606039124429117 ) ) ;
#41877=CARTESIAN_POINT ( 'NONE',  ( -40.53070915468340019, -298.6624442500717009, -197.3162103618080891 ) ) ;
#41878=CARTESIAN_POINT ( 'NONE',  ( -93.54406556422443941, -294.4569962302094837, -317.8850560523690660 ) ) ;
#41880=CARTESIAN_POINT ( 'NONE',  ( -99.38196549910016131, -279.6495326459144621, -224.8357777372608837 ) ) ;
#41881=CARTESIAN_POINT ( 'NONE',  ( 32.89843655600366645, -275.9822301287650816, -290.2896039483050572 ) ) ;
#41882=CARTESIAN_POINT ( 'NONE',  ( -32.32194196038565792, -284.7990067571389545, -194.0060404334572866 ) ) ;
#41883=CARTESIAN_POINT ( 'NONE',  ( -107.3102321367805416, -274.9051788823219908, -243.2105324511977642 ) ) ;
#41885=CARTESIAN_POINT ( 'NONE',  ( 33.86984322072535747, -286.5277573782993272, -253.5284509875894230 ) ) ;
#41886=CARTESIAN_POINT ( 'NONE',  ( -90.18153463057848285, -277.5326517656418446, -218.4625902907441457 ) ) ;
#41887=CARTESIAN_POINT ( 'NONE',  ( -81.62812457132237398, -278.0109564714315411, -211.5256579711591769 ) ) ;
#41888=CARTESIAN_POINT ( 'NONE',  ( -81.49962851721817003, -281.7375843010298695, -330.3534847119999540 ) ) ;
#41889=CARTESIAN_POINT ( 'NONE',  ( 20.66213241999287575, -288.8966279077454828, -222.7960340271066286 ) ) ;
#41890=CARTESIAN_POINT ( 'NONE',  ( -70.61918831324051382, -278.7062861809214382, -335.7808343228430772 ) ) ;
#41892=CARTESIAN_POINT ( 'NONE',  ( -101.5180298370174796, -293.0735131249141432, -231.4485713819197485 ) ) ;
#41893=CARTESIAN_POINT ( 'NONE',  ( -23.15042539779668118, -275.1130522489181089, -345.0643143919090789 ) ) ;
#41894=CARTESIAN_POINT ( 'NONE',  ( 35.45627300659815972, -276.2912953246813572, -277.0205305308269317 ) ) ;
#41895=CARTESIAN_POINT ( 'NONE',  ( 37.80664170710721095, -283.5106728994605305, -267.1106326446460457 ) ) ;
#41897=CARTESIAN_POINT ( 'NONE',  ( 33.72658272043302929, -289.8043227270357534, -296.1769489249382445 ) ) ;
#41898=CARTESIAN_POINT ( 'NONE',  ( -112.3908556221205544, -294.5593570887893975, -269.7871270381273803 ) ) ;
#41900=CARTESIAN_POINT ( 'NONE',  ( 5.477575510487311838, -273.3299939084214998, -210.5675373881622932 ) ) ;
#41901=CARTESIAN_POINT ( 'NONE',  ( 36.87585445388072714, -291.7332972146494967, -273.5655249357238858 ) ) ;
#41902=CARTESIAN_POINT ( 'NONE',  ( 24.80950920047307307, -22.49099280560490399, -345.4124233396505019 ) ) ;
#41904=CARTESIAN_POINT ( 'NONE',  ( -47.63056831016412218, -290.4036346126384274, -194.6979755647244303 ) ) ;
#41905=CARTESIAN_POINT ( 'NONE',  ( -85.36711489528526897, -285.3292034701503326, -326.3968204372601463 ) ) ;
#41906=CARTESIAN_POINT ( 'NONE',  ( 15.60932666036774386, -285.0288925818903749, -215.8619182235494804 ) ) ;
#41907=CARTESIAN_POINT ( 'NONE',  ( -75.03740207644374038, -286.9645654988524370, -207.1597811948694527 ) ) ;
#41908=CARTESIAN_POINT ( 'NONE',  ( -94.25409117056919683, -286.0039061796629198, -224.3675546153488085 ) ) ;
#41909=CARTESIAN_POINT ( 'NONE',  ( -80.99843655355134331, -293.4423891886222577, -208.9404686464075098 ) ) ;
#41910=CARTESIAN_POINT ( 'NONE',  ( 0.3078932788897342787, -274.6350367119741804, -335.9324573039849042 ) ) ;
#41911=CARTESIAN_POINT ( 'NONE',  ( -11.86917589862481570, -277.0628490104348884, -343.0592690511407454 ) ) ;
#41912=CARTESIAN_POINT ( 'NONE',  ( -98.03308049333863039, -289.2420431318808483, -225.3297805556749438 ) ) ;
#41913=CARTESIAN_POINT ( 'NONE',  ( -54.13124844823479975, -277.2618680714534207, -345.5630208357262632 ) ) ;
#41914=CARTESIAN_POINT ( 'NONE',  ( -31.44788545383180889, -296.9573954717786251, -344.8241182409000203 ) ) ;
#41917=CARTESIAN_POINT ( 'NONE',  ( -109.9053897566342499, -283.3906862479408915, -258.6301455001369618 ) ) ;
#41919=CARTESIAN_POINT ( 'NONE',  ( -85.50047368505818213, -277.3865062857793191, -212.7979408751504593 ) ) ;
#41922=CARTESIAN_POINT ( 'NONE',  ( -38.32884969992191770, -272.5198731679579964, -194.0608342937703696 ) ) ;
#41923=CARTESIAN_POINT ( 'NONE',  ( -21.63920055035339018, -276.1942183734960281, -341.8087288914282453 ) ) ;
#41924=CARTESIAN_POINT ( 'NONE',  ( 31.23782842602319221, -295.4312339739874460, -297.4740760878866013 ) ) ;
#41925=CARTESIAN_POINT ( 'NONE',  ( 30.45500933927811005, -280.0064373228339036, -234.3995908357573512 ) ) ;
#41926=CARTESIAN_POINT ( 'NONE',  ( -94.95112746176029361, -296.8578235159841370, -315.5779547936736549 ) ) ;
#41927=CARTESIAN_POINT ( 'NONE',  ( 1.533372733041707958, -295.8590270837037224, -336.2551767639329796 ) ) ;
#41928=CARTESIAN_POINT ( 'NONE',  ( -96.88150751432041830, -296.9752630237763356, -228.1235595667913856 ) ) ;
#41929=CARTESIAN_POINT ( 'NONE',  ( -106.5584265348968529, -292.9309371318239528, -241.3460153535657184 ) ) ;
#41930=CARTESIAN_POINT ( 'NONE',  ( -93.92117932652872980, -285.4306092939054338, -218.0549869248505956 ) ) ;
#41931=CARTESIAN_POINT ( 'NONE',  ( 21.80912381269400058, -273.0470448052685697, -222.9962066773518359 ) ) ;
#41932=CARTESIAN_POINT ( 'NONE',  ( -26.61900576794774054, -286.0181514389761901, -194.0578724827441874 ) ) ;
#41933=CARTESIAN_POINT ( 'NONE',  ( -39.77965525347264020, -282.0013032815086831, -195.7433354173287512 ) ) ;
#41934=CARTESIAN_POINT ( 'NONE',  ( 2.585298234370239090, -285.6608861773589751, -208.9669549900454513 ) ) ;
#41935=CARTESIAN_POINT ( 'NONE',  ( -54.08068690888060104, -287.2667779909892261, -343.5225992571189408 ) ) ;
#41936=CARTESIAN_POINT ( 'NONE',  ( -92.83893396777953910, -239.1568807800618686, -338.3566629249717153 ) ) ;
#41937=CARTESIAN_POINT ( 'NONE',  ( -22.44116389277090917, -285.7556263887379373, -198.7832360582742410 ) ) ;
#41939=CARTESIAN_POINT ( 'NONE',  ( -0.4778688367892073852, -283.5157583794382958, -337.7100911827484993 ) ) ;
#41940=CARTESIAN_POINT ( 'NONE',  ( -84.11346918569235243, -290.4859367224390212, -209.4235973339414443 ) ) ;
#41941=CARTESIAN_POINT ( 'NONE',  ( -101.2317039163527426, -280.7044450471170762, -228.7384085576266557 ) ) ;
#41942=CARTESIAN_POINT ( 'NONE',  ( -111.9247549951099501, -280.0819143946588383, -253.3121824743580532 ) ) ;
#41943=CARTESIAN_POINT ( 'NONE',  ( 35.03307748140585431, -281.2547469748348590, -260.4515029785027309 ) ) ;
#41944=CARTESIAN_POINT ( 'NONE',  ( 14.87123209026071535, -276.7882957706938782, -216.5205166084354858 ) ) ;
#41945=CARTESIAN_POINT ( 'NONE',  ( -32.01250978761930810, -294.9866973648014437, -347.1897338214240563 ) ) ;
#41946=CARTESIAN_POINT ( 'NONE',  ( -100.2410300335867817, -288.0285807071863360, -310.5546634766658940 ) ) ;
#41947=CARTESIAN_POINT ( 'NONE',  ( -78.13310918154785156, -294.5348827684800881, -331.3345653198613263 ) ) ;
#41949=CARTESIAN_POINT ( 'NONE',  ( 10.85937363433953706, -284.3000377125366072, -327.1560846676737810 ) ) ;
#41950=CARTESIAN_POINT ( 'NONE',  ( -107.8549698101690808, -296.4699687175842087, -251.3401685275310058 ) ) ;
#41951=CARTESIAN_POINT ( 'NONE',  ( 39.40228548394804875, -294.6310100162099843, -270.2964404024463647 ) ) ;
#41952=CARTESIAN_POINT ( 'NONE',  ( -48.33583839450611919, -283.8472040996707619, -342.6315932246827742 ) ) ;
#41953=CARTESIAN_POINT ( 'NONE',  ( -1.401012977857417185, -273.5757196555520636, -202.5298035277165241 ) ) ;
#41954=CARTESIAN_POINT ( 'NONE',  ( -111.4415249420204503, -290.9456895251522610, -290.9166220954808750 ) ) ;
#41955=CARTESIAN_POINT ( 'NONE',  ( -37.94839629985712293, -284.1842174689621174, -194.5987433871758583 ) ) ;
#41956=CARTESIAN_POINT ( 'NONE',  ( -105.9871784207898742, -291.3353689238521724, -235.4076355378543894 ) ) ;
#41957=CARTESIAN_POINT ( 'NONE',  ( 24.96655473593886754, -287.3609803330804198, -232.2852875578358010 ) ) ;
#41960=CARTESIAN_POINT ( 'NONE',  ( 84.74214838284052576, 81.45383407810274434, -298.7931483813066507 ) ) ;
#41961=CARTESIAN_POINT ( 'NONE',  ( 21.99644242613736367, -283.7215959280204629, -318.3576993332041525 ) ) ;
#41962=CARTESIAN_POINT ( 'NONE',  ( 35.77081079830085031, -279.2666405000204009, -287.0812184334320705 ) ) ;
#41964=CARTESIAN_POINT ( 'NONE',  ( -72.26490900774759041, -278.4988606263323163, -205.9049657880165967 ) ) ;
#41965=CARTESIAN_POINT ( 'NONE',  ( -5.297447172730779030, -276.3086070062365707, -340.3533328651019474 ) ) ;
#41966=CARTESIAN_POINT ( 'NONE',  ( -112.1108829561311069, -280.5124506622398712, -273.4591371667618773 ) ) ;
#41967=CARTESIAN_POINT ( 'NONE',  ( -96.92303018069374332, -248.0440586835610759, -332.3996513594258317 ) ) ;
#41968=CARTESIAN_POINT ( 'NONE',  ( -5.175390555506203860, -279.0420206143805899, -201.0506943540317479 ) ) ;
#41969=CARTESIAN_POINT ( 'NONE',  ( -68.20526823414608941, -283.6648983628518863, -202.3957814513628932 ) ) ;
#41970=CARTESIAN_POINT ( 'NONE',  ( -94.81950335412450670, -298.9932702060419274, -220.5806862762501623 ) ) ;
#41971=CARTESIAN_POINT ( 'NONE',  ( 33.50727149462049681, -294.2798027013412252, -288.2052111746689889 ) ) ;
#41973=CARTESIAN_POINT ( 'NONE',  ( -72.85062871364783632, -290.2564973392907746, -205.9583113522526219 ) ) ;
#41974=CARTESIAN_POINT ( 'NONE',  ( 15.95041519588032841, -275.4353468568287440, -214.9240975839217640 ) ) ;
#41975=CARTESIAN_POINT ( 'NONE',  ( -65.81314604114456301, -273.6690131771414372, -203.1422458734602117 ) ) ;
#41978=DIRECTION ( 'NONE',  ( -1.000000000000000000, -0.000000000000000000, -0.000000000000000000 ) ) ;
#41980=CARTESIAN_POINT ( 'NONE',  ( 35.82754170954765982, -282.5723709375300245, -265.8347373353341254 ) ) ;
#41981=CARTESIAN_POINT ( 'NONE',  ( -56.32544983727824928, -281.5710994409631098, -196.7297259328687744 ) ) ;
#41982=CARTESIAN_POINT ( 'NONE',  ( -94.47608406517130675, -282.9653463255980910, -316.1966870901869697 ) ) ;
#41983=CARTESIAN_POINT ( 'NONE',  ( -46.63417465790233507, -281.7935173203842396, -196.6578400377112530 ) ) ;
#41984=CARTESIAN_POINT ( 'NONE',  ( 25.96134958546090488, -274.5458729936648297, -308.0895111145813416 ) ) ;
#41987=CARTESIAN_POINT ( 'NONE',  ( -54.08607961464261393, -278.0645714637532251, -345.4075389757854282 ) ) ;
#41991=CARTESIAN_POINT ( 'NONE',  ( -73.46486226879098069, -285.5084218535164950, -336.5519544734756892 ) ) ;
#41992=CARTESIAN_POINT ( 'NONE',  ( 8.958918719834645827, -291.9032233439606330, -213.6486487599679265 ) ) ;
#41993=CARTESIAN_POINT ( 'NONE',  ( 18.56500581520394633, -287.6227629015178309, -323.1602942747457519 ) ) ;
#41994=CARTESIAN_POINT ( 'NONE',  ( -42.72578242040736995, -284.2231796829869950, -196.5310720479739643 ) ) ;
#41995=CARTESIAN_POINT ( 'NONE',  ( -57.53881849520140435, -284.3611245330838528, -199.5447370108839777 ) ) ;
#41996=CARTESIAN_POINT ( 'NONE',  ( -53.65336685484921020, -287.5041829092231183, -342.5546325075417258 ) ) ;
#41997=CARTESIAN_POINT ( 'NONE',  ( 28.51409099227173272, -283.1953442102738450, -302.8824520391976876 ) ) ;
#41998=CARTESIAN_POINT ( 'NONE',  ( 3.788222921563208612, -272.6051628098734909, -207.5832207573302810 ) ) ;
#41999=CARTESIAN_POINT ( 'NONE',  ( -54.76172544957044863, -284.2317206339737368, -196.1790235716186430 ) ) ;
#42000=CARTESIAN_POINT ( 'NONE',  ( -36.93678113737666990, -300.0573775642432679, -195.3609712150442306 ) ) ;
#42001=CARTESIAN_POINT ( 'NONE',  ( -86.53051407642091419, -283.3709929069373743, -213.4548401910015798 ) ) ;
#42002=CARTESIAN_POINT ( 'NONE',  ( -57.18845146303002736, -280.7309636367400003, -199.8663315871593511 ) ) ;
#42003=CARTESIAN_POINT ( 'NONE',  ( 22.38871256499044193, -288.9287967997583451, -224.7077295684182445 ) ) ;
#42006=CARTESIAN_POINT ( 'NONE',  ( 14.43331700338484502, -294.6931859882693061, -215.2560209799082429 ) ) ;
#42007=CARTESIAN_POINT ( 'NONE',  ( -72.61677874022292656, -275.5189877917511012, -336.5622321948986837 ) ) ;
#42008=CARTESIAN_POINT ( 'NONE',  ( -93.48182401163136035, -289.0317140774898235, -322.9015643338077552 ) ) ;
#42009=CARTESIAN_POINT ( 'NONE',  ( -18.03057504029044722, -293.1988835312152446, -341.5897699496218820 ) ) ;
#42010=CARTESIAN_POINT ( 'NONE',  ( -41.05949469224684378, -278.6892064019946247, -196.9620615692227545 ) ) ;
#42011=CARTESIAN_POINT ( 'NONE',  ( -74.98078798095811237, -271.6269403856402391, -206.0782649918740503 ) ) ;
#42012=CARTESIAN_POINT ( 'NONE',  ( 33.59708217105109185, -295.1199185804352396, -289.6166278810821950 ) ) ;
#42013=CARTESIAN_POINT ( 'NONE',  ( 35.77081079830085031, -289.8376638359844719, -253.6410175316879361 ) ) ;
#42014=CARTESIAN_POINT ( 'NONE',  ( -100.9608510622046396, -295.5915997388620440, -228.2028894894580731 ) ) ;
#42015=CARTESIAN_POINT ( 'NONE',  ( -13.00504929679409116, -290.3307013512223307, -340.0329762955774413 ) ) ;
#42016=CARTESIAN_POINT ( 'NONE',  ( 16.78376262359265425, -291.0491589107470531, -216.9540078373960910 ) ) ;
#42017=CARTESIAN_POINT ( 'NONE',  ( -101.6473357735172840, -292.4639642137094029, -234.4770846594436193 ) ) ;
#42019=CARTESIAN_POINT ( 'NONE',  ( -101.2697393067074785, -291.8416246946439969, -234.6788492769836978 ) ) ;
#42022=CARTESIAN_POINT ( 'NONE',  ( -99.53884922450360762, -291.1611827008999853, -315.0996158264422888 ) ) ;
#42023=CARTESIAN_POINT ( 'NONE',  ( 37.23968221855819394, -279.7099127654923336, -281.1325714673180300 ) ) ;
#42024=CARTESIAN_POINT ( 'NONE',  ( 21.80470881790645521, -292.9533294582095095, -227.5531542952972472 ) ) ;
#42025=CARTESIAN_POINT ( 'NONE',  ( 24.59174256752283227, -280.9441236267071531, -224.6090833188391400 ) ) ;
#42026=CARTESIAN_POINT ( 'NONE',  ( 34.30630027885666777, -280.8602972240879581, -242.0676377927984788 ) ) ;
#42027=CARTESIAN_POINT ( 'NONE',  ( -31.75939365461977104, -286.9815068654440893, -345.0378491626451023 ) ) ;
#42028=CARTESIAN_POINT ( 'NONE',  ( 21.50943443380162989, -279.0653299630772040, -225.0921397182632688 ) ) ;
#42030=CARTESIAN_POINT ( 'NONE',  ( -35.17968537688549446, -284.0791100073068947, -195.3794803803363038 ) ) ;
#42031=CARTESIAN_POINT ( 'NONE',  ( -36.73841714686708571, -278.5394898503541299, -194.0439052400876676 ) ) ;
#42032=CARTESIAN_POINT ( 'NONE',  ( -68.36306966320466927, -284.5744498255943995, -200.2100262135897992 ) ) ;
#42033=CARTESIAN_POINT ( 'NONE',  ( 20.80365377746020883, -275.7316505180644981, -225.9364515393609736 ) ) ;
#42035=CARTESIAN_POINT ( 'NONE',  ( -9.443748522189213901, -294.0229316460628297, -201.9829288310226900 ) ) ;
#42036=CARTESIAN_POINT ( 'NONE',  ( 38.14266781216138469, -276.8268595040063360, -258.4145068128436264 ) ) ;
#42037=CARTESIAN_POINT ( 'NONE',  ( -85.12228183661055425, -277.3997901489917695, -325.6467889821460631 ) ) ;
#42038=CARTESIAN_POINT ( 'NONE',  ( -106.0050719069330967, -291.1687945960239290, -235.3961465443591692 ) ) ;
#42039=CARTESIAN_POINT ( 'NONE',  ( 3.741840187476821011, -280.5841742682672475, -333.8379039944675242 ) ) ;
#42040=CARTESIAN_POINT ( 'NONE',  ( -101.3234253852497204, -290.0978208675721248, -234.6234748633722518 ) ) ;
#42041=CARTESIAN_POINT ( 'NONE',  ( -34.94475575749886787, -293.0218790351939901, -345.3228102614483532 ) ) ;
#42042=ORIENTED_EDGE ( 'NONE', *, *, #7316, .T. ) ;
#42044=CARTESIAN_POINT ( 'NONE',  ( -7.239167516334062746, -291.9656571399365248, -203.7891571266743256 ) ) ;
#42047=CARTESIAN_POINT ( 'NONE',  ( 27.36219212280433055, -278.6237833571632905, -239.2376011013261916 ) ) ;
#42048=CARTESIAN_POINT ( 'NONE',  ( -87.30001534795461282, -296.4344745822299956, -212.0073767418146531 ) ) ;
#42049=CARTESIAN_POINT ( 'NONE',  ( 28.22961642614604472, -279.1901131627832910, -232.4044594910565422 ) ) ;
#42050=CARTESIAN_POINT ( 'NONE',  ( -110.2107022552328743, -285.5718615468011876, -293.7153783079858158 ) ) ;
#42051=CARTESIAN_POINT ( 'NONE',  ( -12.01999254973419085, -286.2244361981587986, -201.8935261611792669 ) ) ;
#42052=CARTESIAN_POINT ( 'NONE',  ( 35.39465542970469158, -277.2310034248228021, -282.5076081247422621 ) ) ;
#42053=CARTESIAN_POINT ( 'NONE',  ( -61.57036041639354096, -293.3884373128452694, -341.0191559482328785 ) ) ;
#42054=CARTESIAN_POINT ( 'NONE',  ( -108.9442868164720579, -298.0677189211679661, -289.1473247931770061 ) ) ;
#42055=CARTESIAN_POINT ( 'NONE',  ( 19.47929614660065667, -275.0015746348555012, -316.8406299265187727 ) ) ;
#42058=CARTESIAN_POINT ( 'NONE',  ( -101.6129552175586497, -295.6605510865146584, -312.8243787881069693 ) ) ;
#42059=CARTESIAN_POINT ( 'NONE',  ( 35.39801062582398572, -289.2676602293741439, -254.5418676521328791 ) ) ;
#42061=CARTESIAN_POINT ( 'NONE',  ( -37.25958740186422347, -289.7025121495771600, -343.4630052775654576 ) ) ;
#42063=CARTESIAN_POINT ( 'NONE',  ( -77.35959418939796706, -278.5884135566461168, -204.7908966724019137 ) ) ;
#42064=CARTESIAN_POINT ( 'NONE',  ( -82.91684607929566653, -298.0986064139047471, -208.3577355048848858 ) ) ;
#42065=CARTESIAN_POINT ( 'NONE',  ( -112.1443741957517233, -288.5387581724811525, -282.3971236965435878 ) ) ;
#42066=CARTESIAN_POINT ( 'NONE',  ( -70.79484542062520802, -295.8146109541293072, -339.7054972979488525 ) ) ;
#42067=CARTESIAN_POINT ( 'NONE',  ( 10.94160792830293261, -293.0751463410686597, -215.5140034193332497 ) ) ;
#42071=CARTESIAN_POINT ( 'NONE',  ( -23.41926306724479900, -290.3975307037973721, -345.4405661913328345 ) ) ;
#42072=CARTESIAN_POINT ( 'NONE',  ( -37.37352853689063181, -276.5519495502701375, -190.3611179825600175 ) ) ;
#42073=CARTESIAN_POINT ( 'NONE',  ( 28.21375987243529337, -281.4277882269954603, -310.6589574306599957 ) ) ;
#42074=CARTESIAN_POINT ( 'NONE',  ( -26.45141992758102845, -284.9135586063146661, -344.4503898334593259 ) ) ;
#42075=CARTESIAN_POINT ( 'NONE',  ( -1.231864890178082872, -285.0964021877157961, -203.0210400719131201 ) ) ;
#42076=CARTESIAN_POINT ( 'NONE',  ( -110.8448092849325093, -288.4786531565889049, -282.2146085632067525 ) ) ;
#42077=CARTESIAN_POINT ( 'NONE',  ( 35.39325635673228732, -277.1401082105775231, -248.9663918718121636 ) ) ;
#42078=VERTEX_POINT ( 'NONE', #48648 ) ;
#42079=CARTESIAN_POINT ( 'NONE',  ( -108.6067547304953962, -278.7615401045008525, -254.4832753974120578 ) ) ;
#42080=CARTESIAN_POINT ( 'NONE',  ( 18.91986168076719466, -280.2395298437859310, -223.6669689975476274 ) ) ;
#42081=CARTESIAN_POINT ( 'NONE',  ( 8.069140569896507742, -277.5275090555168731, -332.2277495529352223 ) ) ;
#42082=CARTESIAN_POINT ( 'NONE',  ( -48.04802613618277718, -278.7139081193637367, -194.4564924471395670 ) ) ;
#42083=CARTESIAN_POINT ( 'NONE',  ( 195.1507973710101567, 283.8842776367829401, -110.7649439234235729 ) ) ;
#42084=CARTESIAN_POINT ( 'NONE',  ( -70.04246372125138009, -274.5731428576596045, -200.8954679847426519 ) ) ;
#42085=CARTESIAN_POINT ( 'NONE',  ( -103.6368475773368942, -274.5686611828822947, -232.4706282480738935 ) ) ;
#42086=CARTESIAN_POINT ( 'NONE',  ( -69.91165696735023971, -282.1233781216988064, -202.8022627189028810 ) ) ;
#42090=CARTESIAN_POINT ( 'NONE',  ( 34.82840873836469342, -288.8009209392869820, -283.2336259117558939 ) ) ;
#42091=CARTESIAN_POINT ( 'NONE',  ( -110.7482355669279315, -286.5636539579506916, -250.5301347197553810 ) ) ;
#42092=CARTESIAN_POINT ( 'NONE',  ( 27.11643658544443625, -287.3714257439831954, -304.9513084693872997 ) ) ;
#42093=CARTESIAN_POINT ( 'NONE',  ( -113.5393281124190707, -283.9217793124122409, -281.3888541548994908 ) ) ;
#42094=CARTESIAN_POINT ( 'NONE',  ( 22.77689436350958374, -279.3605917052735776, -227.5569708410353371 ) ) ;
#42095=CARTESIAN_POINT ( 'NONE',  ( -33.19292430996794963, -287.9652290802163748, -196.1912722001160034 ) ) ;
#42096=CARTESIAN_POINT ( 'NONE',  ( 29.93963459380002945, -280.4345705094478944, -300.5517617227233700 ) ) ;
#42097=CARTESIAN_POINT ( 'NONE',  ( -83.30220137022500637, -279.0119753137107068, -327.7753249892749636 ) ) ;
#42098=CARTESIAN_POINT ( 'NONE',  ( 27.91343983204256674, -275.5988971401802132, -237.5014900138333189 ) ) ;
#42099=CARTESIAN_POINT ( 'NONE',  ( 33.66844956706929537, -286.7153623773274944, -299.2350239973816315 ) ) ;
#42100=CARTESIAN_POINT ( 'NONE',  ( -67.80790689833449392, -284.2447944517442693, -340.9016670723125912 ) ) ;
#42101=CARTESIAN_POINT ( 'NONE',  ( -106.9473036443437906, -284.6242651026552153, -303.1420097061146635 ) ) ;
#42102=CARTESIAN_POINT ( 'NONE',  ( -6.031017544437445643, -282.7955433783161538, -336.3190961069706759 ) ) ;
#42105=CARTESIAN_POINT ( 'NONE',  ( -112.3417001280820386, -272.5521521680024648, -270.3611179825637691 ) ) ;
#42106=CARTESIAN_POINT ( 'NONE',  ( -43.06497225699423836, -290.9840985263101061, -345.9094444818704233 ) ) ;
#42107=CARTESIAN_POINT ( 'NONE',  ( -56.05186982195797185, -290.5010254134408569, -196.1227815674955650 ) ) ;
#42108=CARTESIAN_POINT ( 'NONE',  ( -85.45575128015269684, -272.4266123007801070, -215.0807985892640488 ) ) ;
#42109=CARTESIAN_POINT ( 'NONE',  ( 29.48197768727347068, -293.3967643590737566, -308.5200631123209973 ) ) ;
#42110=CARTESIAN_POINT ( 'NONE',  ( -104.6891480445574985, -288.6315859034411346, -300.4042494969926906 ) ) ;
#42111=CARTESIAN_POINT ( 'NONE',  ( -6.832337385176574962, -290.6980681784572766, -202.9285383130988976 ) ) ;
#42112=CARTESIAN_POINT ( 'NONE',  ( -10.56501337521648587, -289.9001132167441597, -338.7540531596937967 ) ) ;
#42114=CARTESIAN_POINT ( 'NONE',  ( -90.17118355432761234, -291.7987423681811947, -323.6699113191148172 ) ) ;
#42115=CARTESIAN_POINT ( 'NONE',  ( -98.52363673168103730, -289.1445077760039908, -226.6942076087616158 ) ) ;
#42116=CARTESIAN_POINT ( 'NONE',  ( -45.51933279605668758, -293.9488161272667526, -195.7571921396720995 ) ) ;
#42117=CARTESIAN_POINT ( 'NONE',  ( 11.28135300780948214, -287.6865909179635423, -215.5279746838696440 ) ) ;
#42118=CARTESIAN_POINT ( 'NONE',  ( -4.154314380642599502, -294.4888015521621014, -202.9034280918289426 ) ) ;
#42121=CARTESIAN_POINT ( 'NONE',  ( 33.17353357999118657, -277.1885329724655662, -243.7902953377071071 ) ) ;
#42122=CARTESIAN_POINT ( 'NONE',  ( -92.58802361285535198, -295.0162071209260830, -323.7652616586175327 ) ) ;
#42123=CARTESIAN_POINT ( 'NONE',  ( -33.97242895344523106, -272.3349687238520573, -196.4245098187130338 ) ) ;
#42124=CARTESIAN_POINT ( 'NONE',  ( -90.12378267622244721, -275.8847210037165496, -322.9259199327958072 ) ) ;
#42125=CARTESIAN_POINT ( 'NONE',  ( -34.03807967223432485, -275.2997065238326400, -197.0384298331000537 ) ) ;
#42127=CARTESIAN_POINT ( 'NONE',  ( -69.96912571342598142, -296.9159226804785021, -336.3219095078279679 ) ) ;
#42129=DIRECTION ( 'NONE',  ( -1.000000000000000000, -0.000000000000000000, -0.000000000000000000 ) ) ;
#42130=CARTESIAN_POINT ( 'NONE',  ( -72.93436184399428157, -298.3704235147003487, -206.4411355109402564 ) ) ;
#42132=CARTESIAN_POINT ( 'NONE',  ( 36.93986834925429008, -285.4093115655298334, -257.6100704862456041 ) ) ;
#42133=CARTESIAN_POINT ( 'NONE',  ( -44.56908489952338925, -297.9582964478407234, -197.6693916683557006 ) ) ;
#42134=CARTESIAN_POINT ( 'NONE',  ( -32.30641958262449975, -286.1139684545679529, -193.5127647814072986 ) ) ;
#42135=CARTESIAN_POINT ( 'NONE',  ( -99.01474309014216146, -289.6055843361505708, -316.4500430296726563 ) ) ;
#42136=CARTESIAN_POINT ( 'NONE',  ( -105.6642417930441837, -298.1163139150809798, -302.1484912650414003 ) ) ;
#42137=CARTESIAN_POINT ( 'NONE',  ( 9.352746220141005651, -292.4090604623286822, -328.9055307825724981 ) ) ;
#42138=CARTESIAN_POINT ( 'NONE',  ( -45.24656889051706798, -279.1517471477288268, -193.8774083148039153 ) ) ;
#42139=CARTESIAN_POINT ( 'NONE',  ( -85.28047601435908120, -294.9094976428776249, -210.1954327657594206 ) ) ;
#42141=CARTESIAN_POINT ( 'NONE',  ( -88.95111478276238870, -288.5924118681971322, -322.5492279637877004 ) ) ;
#42143=CARTESIAN_POINT ( 'NONE',  ( -88.10121063534423058, -287.7618270281723198, -325.6445708824180088 ) ) ;
#42144=CARTESIAN_POINT ( 'NONE',  ( -98.42867341926329061, -274.6408742057246855, -229.0500343712124618 ) ) ;
#42145=CARTESIAN_POINT ( 'NONE',  ( -53.65253667913266611, -281.2722276150786342, -195.6573632819490172 ) ) ;
#42146=CARTESIAN_POINT ( 'NONE',  ( -90.45789314581270446, -295.3245937662110805, -216.9094871293813753 ) ) ;
#42147=CARTESIAN_POINT ( 'NONE',  ( 35.35234721594390095, -281.4570432862635698, -263.1513449924633505 ) ) ;
#42148=CARTESIAN_POINT ( 'NONE',  ( -112.6047098731618803, -296.5154422344219824, -286.6239396518015496 ) ) ;
#42149=CARTESIAN_POINT ( 'NONE',  ( -36.49258129533864548, -299.5830937490768520, -196.6675549952466611 ) ) ;
#42151=CARTESIAN_POINT ( 'NONE',  ( 35.04776516096256955, -283.2995422298061499, -250.6970259347930892 ) ) ;
#42153=CARTESIAN_POINT ( 'NONE',  ( -101.6797210199117387, -295.1349046563659613, -305.3472225843132719 ) ) ;
#42156=CARTESIAN_POINT ( 'NONE',  ( -15.63054467777635992, -284.7497122728523777, -341.7787105588999452 ) ) ;
#42158=CARTESIAN_POINT ( 'NONE',  ( -85.28047601435909542, -294.9094976428776818, -210.1954327657594206 ) ) ;
#42159=CARTESIAN_POINT ( 'NONE',  ( 34.03046139196352726, -275.1128073459044003, -298.9680657569005575 ) ) ;
#42160=CARTESIAN_POINT ( 'NONE',  ( 27.48751066261156595, -292.9291070127144962, -236.8026103765939467 ) ) ;
#42161=CARTESIAN_POINT ( 'NONE',  ( 34.91428985651987915, -283.2623752425332100, -284.9084766489496587 ) ) ;
#42163=CARTESIAN_POINT ( 'NONE',  ( 34.02092610902858638, -277.3979666706746912, -289.1711151475886936 ) ) ;
#42164=CARTESIAN_POINT ( 'NONE',  ( -83.51261380528107736, -285.0962838659742715, -331.3115024803383903 ) ) ;
#42166=CARTESIAN_POINT ( 'NONE',  ( -83.05394679926037327, -282.4885527937484540, -327.8503918926580241 ) ) ;
#42167=CARTESIAN_POINT ( 'NONE',  ( -102.5632736793492796, -281.0459011237286404, -233.3321159723420806 ) ) ;
#42168=CARTESIAN_POINT ( 'NONE',  ( -113.0686821389476222, -272.8967761882815921, -256.1327989363236952 ) ) ;
#42169=CARTESIAN_POINT ( 'NONE',  ( 24.48113922993194436, -274.7751614573199390, -224.4597395910907665 ) ) ;
#42171=CARTESIAN_POINT ( 'NONE',  ( 15.35257030271881362, -296.2211767302954968, -323.0133506394817573 ) ) ;
#42172=CYLINDRICAL_SURFACE ( 'NONE', #53614, 2.397123461337413719 ) ;
#42174=CARTESIAN_POINT ( 'NONE',  ( -89.87300498813381466, -293.9233782169240499, -325.0297771315518389 ) ) ;
#42175=CARTESIAN_POINT ( 'NONE',  ( 32.95535355670186561, -275.3233093522191552, -290.3144907837802293 ) ) ;
#42176=CARTESIAN_POINT ( 'NONE',  ( -27.81502623903721982, -296.4535314705951805, -346.1235756325683042 ) ) ;
#42177=CARTESIAN_POINT ( 'NONE',  ( 39.10700906647314667, -294.8280454373270345, -275.9945798117737468 ) ) ;
#42178=CARTESIAN_POINT ( 'NONE',  ( 22.65831315928593170, -290.1646338485070373, -315.1042372017852244 ) ) ;
#42179=CARTESIAN_POINT ( 'NONE',  ( -111.7872645182141156, -276.6562656011413992, -262.2578052085316358 ) ) ;
#42180=CARTESIAN_POINT ( 'NONE',  ( -104.4181645627269006, -280.0426010191475257, -302.7612964063426944 ) ) ;
#42181=CARTESIAN_POINT ( 'NONE',  ( -98.37783157152060198, -294.0493405247094074, -312.9745531562338670 ) ) ;
#42182=CARTESIAN_POINT ( 'NONE',  ( 36.35255977281524764, -283.6368109510935938, -288.0080504870875870 ) ) ;
#42183=CARTESIAN_POINT ( 'NONE',  ( -33.20753275144534911, -285.0256165265851678, -197.1186374804175045 ) ) ;
#42184=CARTESIAN_POINT ( 'NONE',  ( 27.25360408407748025, -24.20672218296157752, -344.2562845684955164 ) ) ;
#42186=CARTESIAN_POINT ( 'NONE',  ( -104.6153801052060146, -284.6014429029134476, -241.8350534578070210 ) ) ;
#42188=CARTESIAN_POINT ( 'NONE',  ( 36.89605633750436908, -282.8736171719617118, -289.6029480837335655 ) ) ;
#42189=CARTESIAN_POINT ( 'NONE',  ( -109.5976008122744361, -283.6696528231084926, -244.9230847573956567 ) ) ;
#42190=CARTESIAN_POINT ( 'NONE',  ( -112.4896841582854989, -279.6907874466978683, -254.6260255366181582 ) ) ;
#42192=CARTESIAN_POINT ( 'NONE',  ( -71.24524488177144121, -279.0117448326091107, -338.7223453594258444 ) ) ;
#42193=CARTESIAN_POINT ( 'NONE',  ( 12.91927517772756495, -281.3841028665469821, -212.1619156890937745 ) ) ;
#42194=CARTESIAN_POINT ( 'NONE',  ( -105.5937364680635966, -299.2662352645559167, -254.8156830097664738 ) ) ;
#42195=CARTESIAN_POINT ( 'NONE',  ( -113.0732809282716147, -274.2376448861158451, -284.1882621119263490 ) ) ;
#42197=CARTESIAN_POINT ( 'NONE',  ( 22.94335637594691235, -276.9462939732044902, -226.0244470289034950 ) ) ;
#42198=CARTESIAN_POINT ( 'NONE',  ( -104.7838118829956073, -255.6369273504282091, -326.4926257996353343 ) ) ;
#42199=CARTESIAN_POINT ( 'NONE',  ( -49.38295309825753776, -277.9179990950224237, -196.6939270010225300 ) ) ;
#42200=CARTESIAN_POINT ( 'NONE',  ( -110.5594846597458911, -292.0542383915988012, -290.6867186739625595 ) ) ;
#42201=CARTESIAN_POINT ( 'NONE',  ( 28.83431919691496503, -292.4803615584298768, -239.1831744904247898 ) ) ;
#42202=CARTESIAN_POINT ( 'NONE',  ( -87.34920049625704053, -289.2351826819626126, -328.9014072892380796 ) ) ;
#42204=CARTESIAN_POINT ( 'NONE',  ( 1.454508968936686575, -293.1190228977339984, -336.1901423747411286 ) ) ;
#42205=CARTESIAN_POINT ( 'NONE',  ( -57.59457826035073680, -284.1862965901574967, -199.3413116473142566 ) ) ;
#42206=CARTESIAN_POINT ( 'NONE',  ( -107.7502061521683316, -292.7198254812090568, -246.8343723662671891 ) ) ;
#42207=CARTESIAN_POINT ( 'NONE',  ( -16.96173304368145196, -284.7998639787448951, -199.4885245944802534 ) ) ;
#42208=CARTESIAN_POINT ( 'NONE',  ( -45.67889087126178538, -284.4750703068490907, -343.4311843225646612 ) ) ;
#42210=CARTESIAN_POINT ( 'NONE',  ( -99.84645246660110729, -292.0854451413042625, -225.7968256807372143 ) ) ;
#42211=CARTESIAN_POINT ( 'NONE',  ( 5.633343002982027059, -282.9443524922580195, -329.4469378496282275 ) ) ;
#42212=CARTESIAN_POINT ( 'NONE',  ( -34.88283910893213147, -293.8168352204102689, -346.9245735088458105 ) ) ;
#42213=CARTESIAN_POINT ( 'NONE',  ( -59.96994870452659399, -290.1409676069350780, -343.7921821615907447 ) ) ;
#42214=CARTESIAN_POINT ( 'NONE',  ( -98.10714326194072044, -290.4137429133613750, -317.5531493466613711 ) ) ;
#42215=CARTESIAN_POINT ( 'NONE',  ( 34.99584765746132575, -287.5845243074135738, -260.1797802226952285 ) ) ;
#42218=CARTESIAN_POINT ( 'NONE',  ( -98.98942229970184314, -297.8185843613829888, -314.4933335870838960 ) ) ;
#42219=CARTESIAN_POINT ( 'NONE',  ( -73.03554292154213101, -296.2743859815861924, -202.6325172155620749 ) ) ;
#42220=CARTESIAN_POINT ( 'NONE',  ( -107.8415725520628712, -277.8727106818788002, -250.4859891648111159 ) ) ;
#42221=CARTESIAN_POINT ( 'NONE',  ( -94.09562997993657518, -272.7671124503519877, -218.3944026816361372 ) ) ;
#42223=CARTESIAN_POINT ( 'NONE',  ( -96.98081189327255913, -294.4316892329314328, -313.6710468714568378 ) ) ;
#42224=CARTESIAN_POINT ( 'NONE',  ( 32.22176225944927808, -277.6462176144157752, -295.7866218366769999 ) ) ;
#42225=CARTESIAN_POINT ( 'NONE',  ( -106.5595144590962491, -271.0459273630126518, -243.3911021035835631 ) ) ;
#42226=CARTESIAN_POINT ( 'NONE',  ( -26.13170543039678861, -296.1113294050147715, -342.8970850806831550 ) ) ;
#42227=CARTESIAN_POINT ( 'NONE',  ( -50.51330823245528023, -296.3040016795968654, -342.4772383211392253 ) ) ;
#42228=CARTESIAN_POINT ( 'NONE',  ( 133.0872704186301405, -299.5541904835127980, -195.3611179825600175 ) ) ;
#42229=CARTESIAN_POINT ( 'NONE',  ( -102.4216391125737999, -297.6292531184909080, -309.9974896128650812 ) ) ;
#42230=CARTESIAN_POINT ( 'NONE',  ( -111.7824907539996673, -294.6866888240654703, -259.8472399430826272 ) ) ;
#42231=CARTESIAN_POINT ( 'NONE',  ( -7.235835244455974369, -293.1092325283569267, -203.7463330762865041 ) ) ;
#42232=CARTESIAN_POINT ( 'NONE',  ( -114.1806035973878863, -273.3907171491254076, -267.5098654519179036 ) ) ;
#42233=CARTESIAN_POINT ( 'NONE',  ( -87.14137452677120166, -288.3366226459800714, -324.6092932845065206 ) ) ;
#42234=CARTESIAN_POINT ( 'NONE',  ( -86.64354579147382651, -275.3675513877705043, -213.7734863356731694 ) ) ;
#42235=CARTESIAN_POINT ( 'NONE',  ( -95.04447986815924310, -273.7341246248622610, -219.4698995494528333 ) ) ;
#42236=CARTESIAN_POINT ( 'NONE',  ( -106.7282076962837181, -297.1892042104578309, -247.4499622215209911 ) ) ;
#42237=CARTESIAN_POINT ( 'NONE',  ( -38.17750912248671824, -282.0216133365882456, -195.0105491031473548 ) ) ;
#42238=CARTESIAN_POINT ( 'NONE',  ( -17.10620383300768665, -278.9929290163530027, -196.5788507280984163 ) ) ;
#42240=CARTESIAN_POINT ( 'NONE',  ( -41.57183794321338866, -282.4525661027702768, -347.1950050990007526 ) ) ;
#42241=CARTESIAN_POINT ( 'NONE',  ( 29.00381038165020442, -275.4074882379208020, -309.2402386202039679 ) ) ;
#42242=CARTESIAN_POINT ( 'NONE',  ( 34.84459382249985993, -280.2645185754401496, -294.9294596004835398 ) ) ;
#42243=CARTESIAN_POINT ( 'NONE',  ( 5.168896820478852128, -278.6254773600643375, -208.3701704873829499 ) ) ;
#42245=CARTESIAN_POINT ( 'NONE',  ( -72.17070865561098003, -272.1570538325202619, -205.4790794785414221 ) ) ;
#42246=CARTESIAN_POINT ( 'NONE',  ( 35.35380634154680024, -277.7899070664295209, -288.8610073231438946 ) ) ;
#42247=DIRECTION ( 'NONE',  ( -1.000000000000000000, -0.000000000000000000, -0.000000000000000000 ) ) ;
#42249=CARTESIAN_POINT ( 'NONE',  ( -99.90346104626898693, -295.3692772052853002, -227.2105427463845899 ) ) ;
#42250=CARTESIAN_POINT ( 'NONE',  ( -25.25977348276387247, -290.2255582279785813, -195.9807855761962685 ) ) ;
#42251=CARTESIAN_POINT ( 'NONE',  ( -94.71130554120206568, -291.2488173687601716, -219.0022981485447815 ) ) ;
#42252=CARTESIAN_POINT ( 'NONE',  ( 36.14746065538369635, -277.3492191554605029, -254.5088575786688239 ) ) ;
#42253=CARTESIAN_POINT ( 'NONE',  ( -65.29108103802053620, -271.6867263482307067, -200.7496220629793697 ) ) ;
#42255=CARTESIAN_POINT ( 'NONE',  ( -38.68201801359813174, -284.9889888730991174, -345.9092334427348305 ) ) ;
#42257=CARTESIAN_POINT ( 'NONE',  ( -112.3519692451748142, -282.5201479316810946, -272.8408409343114158 ) ) ;
#42259=CARTESIAN_POINT ( 'NONE',  ( -20.77338096908489717, -293.6297602833795395, -341.9160998228068706 ) ) ;
#42260=CARTESIAN_POINT ( 'NONE',  ( 33.86133416336743096, -285.4179608160854968, -249.3163830905704117 ) ) ;
#42263=CARTESIAN_POINT ( 'NONE',  ( -34.24338683495191304, -293.0130252916814015, -345.2970980308921867 ) ) ;
#42264=CARTESIAN_POINT ( 'NONE',  ( -108.3758997270184921, -283.3901913537162613, -242.3454811052901334 ) ) ;
#42265=CARTESIAN_POINT ( 'NONE',  ( -54.70051500970891567, -281.4255993396954523, -198.5789091378471483 ) ) ;
#42266=CARTESIAN_POINT ( 'NONE',  ( -113.0971089942133858, -285.9044788522738259, -258.6474786108802846 ) ) ;
#42267=CARTESIAN_POINT ( 'NONE',  ( 38.60627189909572365, -279.8227406011047265, -272.7858976308131105 ) ) ;
#42268=CARTESIAN_POINT ( 'NONE',  ( 34.99614351355761954, -287.4178711535176376, -260.1818832611007224 ) ) ;
#42269=CARTESIAN_POINT ( 'NONE',  ( -78.95032884280882968, -279.0502580464121820, -331.1199194987961505 ) ) ;
#42270=CARTESIAN_POINT ( 'NONE',  ( -87.19811882456576768, -278.5714949338289443, -323.9049247334257302 ) ) ;
#42273=CARTESIAN_POINT ( 'NONE',  ( -94.58400159273634245, -287.2083764284462291, -221.2754231474131075 ) ) ;
#42275=CARTESIAN_POINT ( 'NONE',  ( -23.35769572636721492, -298.0560261227212777, -193.3614995326353494 ) ) ;
#42276=CARTESIAN_POINT ( 'NONE',  ( 36.38773870376633113, -289.6834478554512202, -282.0967856895698560 ) ) ;
#42278=CARTESIAN_POINT ( 'NONE',  ( -115.3288506153726871, -286.8376638359844719, -288.1938231032136741 ) ) ;
#42280=CARTESIAN_POINT ( 'NONE',  ( 25.41429355638885212, -272.9947051449473179, -228.9882563095496835 ) ) ;
#42282=CARTESIAN_POINT ( 'NONE',  ( 30.18390022370923731, -292.4123690577949901, -305.6702345193893393 ) ) ;
#42283=CARTESIAN_POINT ( 'NONE',  ( -86.13673567776757523, -296.8609934912890935, -215.9825105417341433 ) ) ;
#42284=CARTESIAN_POINT ( 'NONE',  ( 36.32395554261007220, -289.1168641302172659, -273.7728047627415435 ) ) ;
#42285=CARTESIAN_POINT ( 'NONE',  ( 5.491607269823510329, -282.4012247385679188, -210.0015140351610228 ) ) ;
#42286=CARTESIAN_POINT ( 'NONE',  ( -45.94128965665010611, -290.5842973735720989, -346.3391519802719927 ) ) ;
#42287=CARTESIAN_POINT ( 'NONE',  ( -113.8759504293081477, -291.8922074113866074, -268.3842748251791477 ) ) ;
#42288=CARTESIAN_POINT ( 'NONE',  ( -111.4712786417625523, -286.4017563327539051, -282.0868400082505332 ) ) ;
#42289=CARTESIAN_POINT ( 'NONE',  ( -7.538949499501011786, -280.5988727940028866, -199.3482512648447198 ) ) ;
#42291=CARTESIAN_POINT ( 'NONE',  ( 29.61479403485629547, -292.0923948850980310, -305.3774296770954493 ) ) ;
#42292=CARTESIAN_POINT ( 'NONE',  ( 39.71045392701341825, -281.3801105752831404, -269.9323865911590588 ) ) ;
#42293=CARTESIAN_POINT ( 'NONE',  ( 21.64889258855931686, -276.7890627938688226, -225.2738572682821996 ) ) ;
#42295=CARTESIAN_POINT ( 'NONE',  ( 7.399455738971494334, -277.1948066931273047, -214.2051214447836571 ) ) ;
#42297=CARTESIAN_POINT ( 'NONE',  ( 36.91062037888140424, -273.9973579792975329, -286.5639148675630281 ) ) ;
#42299=CARTESIAN_POINT ( 'NONE',  ( 35.09465133165635109, -280.9291323441817099, -260.4472580575271650 ) ) ;
#42300=CARTESIAN_POINT ( 'NONE',  ( -113.8346825827095330, -279.7056499331107489, -274.4638430257937216 ) ) ;
#42301=CIRCLE ( 'NONE', #1484, 3.491568894204821749 ) ;
#42302=CARTESIAN_POINT ( 'NONE',  ( -54.34175520056412978, -275.1443525508907442, -198.8611766951847528 ) ) ;
#42303=CARTESIAN_POINT ( 'NONE',  ( -46.46560637000157357, -284.9977964188837518, -194.1405528607957081 ) ) ;
#42304=CARTESIAN_POINT ( 'NONE',  ( -104.9645617908895616, -291.9113212542195583, -300.5728567032115279 ) ) ;
#42305=CARTESIAN_POINT ( 'NONE',  ( -24.31661036425930433, -275.8157626102602649, -195.2289749244463337 ) ) ;
#42306=CARTESIAN_POINT ( 'NONE',  ( -109.6413436277052540, -274.1847978990736010, -245.3399305201349421 ) ) ;
#42308=CARTESIAN_POINT ( 'NONE',  ( -112.2089796716966106, -298.5734697482130855, -268.7174222125194660 ) ) ;
#42309=CARTESIAN_POINT ( 'NONE',  ( -51.38634014322530419, -281.2318447437779128, -343.9175740812002005 ) ) ;
#42310=CARTESIAN_POINT ( 'NONE',  ( -111.9730258420098323, -290.4555910380806267, -251.4424713074985220 ) ) ;
#42311=CARTESIAN_POINT ( 'NONE',  ( 32.79884400571190639, -273.9067867190649963, -296.0484217280280177 ) ) ;
#42312=CARTESIAN_POINT ( 'NONE',  ( 36.59559386667802983, -288.9192593325754501, -251.9297052691628664 ) ) ;
#42313=CARTESIAN_POINT ( 'NONE',  ( -94.52341181032628015, -290.1183116424578543, -224.4665854958456919 ) ) ;
#42315=CARTESIAN_POINT ( 'NONE',  ( -108.2584001906662365, -288.7630462449582751, -298.8115651460922777 ) ) ;
#42316=CARTESIAN_POINT ( 'NONE',  ( -110.3276322273784444, -290.1721227383386008, -273.9057526129781195 ) ) ;
#42317=ORIENTED_EDGE ( 'NONE', *, *, #23269, .T. ) ;
#42318=CARTESIAN_POINT ( 'NONE',  ( 38.78547465501085867, -288.7537375978986915, -280.0703550040175855 ) ) ;
#42319=CARTESIAN_POINT ( 'NONE',  ( -96.10749623106048034, -278.2778698193772584, -313.7256870808129179 ) ) ;
#42320=CARTESIAN_POINT ( 'NONE',  ( -13.88969348611722943, -293.6751192062753830, -343.3782111430602413 ) ) ;
#42321=CARTESIAN_POINT ( 'NONE',  ( -111.8534275305500074, -284.6428104518091118, -289.7458969499454042 ) ) ;
#42322=CARTESIAN_POINT ( 'NONE',  ( -8.481980394220936859, -282.9969334636175518, -337.4372244864086952 ) ) ;
#42323=CARTESIAN_POINT ( 'NONE',  ( -71.04534101611670849, -196.2794566099099995, -360.5068448367716769 ) ) ;
#42324=CARTESIAN_POINT ( 'NONE',  ( 201.7737866479175750, 295.5635967683617196, -68.54576060224776768 ) ) ;
#42325=CARTESIAN_POINT ( 'NONE',  ( 5.009449089156567503, -58.86080836571535713, -351.0592355680212222 ) ) ;
#42326=CARTESIAN_POINT ( 'NONE',  ( -43.48551367926898337, -273.1698670285560411, -197.4072412621284229 ) ) ;
#42327=CARTESIAN_POINT ( 'NONE',  ( -1.559789011583864404, -273.4586660888683696, -206.3633002098954989 ) ) ;
#42328=CARTESIAN_POINT ( 'NONE',  ( -88.56913578991110114, -295.2554266174283839, -327.8370669536779474 ) ) ;
#42329=CARTESIAN_POINT ( 'NONE',  ( 202.1135227227061364, 289.8103657602464978, -82.43770367997073834 ) ) ;
#42330=CARTESIAN_POINT ( 'NONE',  ( -15.89941324210910167, -273.0085409260970550, -196.8654961622563349 ) ) ;
#42331=CARTESIAN_POINT ( 'NONE',  ( -111.2828678737150057, -298.5054208216035931, -263.2037346356970602 ) ) ;
#42332=CARTESIAN_POINT ( 'NONE',  ( -12.16691537103328180, -293.4671075416617896, -201.4560448007708544 ) ) ;
#42334=CARTESIAN_POINT ( 'NONE',  ( -106.9479631355059013, -297.0778408655646103, -302.7306771767038072 ) ) ;
#42335=CARTESIAN_POINT ( 'NONE',  ( 34.82099056833637007, -288.1961430047854265, -281.8660588170914707 ) ) ;
#42336=CARTESIAN_POINT ( 'NONE',  ( 0.4699689440745843938, -295.3644352029350557, -337.2674955967511892 ) ) ;
#42337=CARTESIAN_POINT ( 'NONE',  ( -50.45086305970222895, -295.7074471055738059, -346.2284531132146981 ) ) ;
#42338=CARTESIAN_POINT ( 'NONE',  ( 31.80035113723905127, -293.4058135548237374, -246.7863298713807012 ) ) ;
#42340=CARTESIAN_POINT ( 'NONE',  ( 27.86581817928561478, -277.9786413101349467, -308.5356350356919393 ) ) ;
#42344=CARTESIAN_POINT ( 'NONE',  ( -114.1708897964509646, -278.0085002865974957, -274.4602054389801538 ) ) ;
#42345=CARTESIAN_POINT ( 'NONE',  ( 32.32569665369121736, -276.7920182781443827, -292.9412480483022136 ) ) ;
#42346=CARTESIAN_POINT ( 'NONE',  ( 30.33745307036346617, -276.8614041650806712, -235.8139584224055341 ) ) ;
#42347=CARTESIAN_POINT ( 'NONE',  ( -96.97068175585063443, -297.7932241403557896, -228.0730910909286138 ) ) ;
#42348=CARTESIAN_POINT ( 'NONE',  ( -110.3916744350586328, -295.0051563750857326, -279.6624581978121569 ) ) ;
#42350=CARTESIAN_POINT ( 'NONE',  ( -113.1768922274226270, -279.2069937476874770, -257.3784163155972919 ) ) ;
#42351=CARTESIAN_POINT ( 'NONE',  ( -48.60574581701071395, -277.3661147383069761, -342.5382392165624879 ) ) ;
#42352=CARTESIAN_POINT ( 'NONE',  ( 37.54428224780750867, -286.0390112312750261, -254.6327574638088151 ) ) ;
#42353=CARTESIAN_POINT ( 'NONE',  ( -86.28822615237660898, -299.3754136867460147, -213.2463084346213122 ) ) ;
#42355=CARTESIAN_POINT ( 'NONE',  ( 3.696748015782929997, -287.6816985566318863, -330.9899108658565297 ) ) ;
#42356=CARTESIAN_POINT ( 'NONE',  ( 14.05469148327361495, -279.0250687541832235, -217.0319533307971653 ) ) ;
#42357=CARTESIAN_POINT ( 'NONE',  ( -43.78473630159547270, -278.5439990237646271, -197.0038471786520233 ) ) ;
#42359=CARTESIAN_POINT ( 'NONE',  ( -47.03146446348424092, -287.9293704560428182, -195.9383397457096123 ) ) ;
#42360=CARTESIAN_POINT ( 'NONE',  ( -61.90834894662256005, -278.5836759167299306, -339.5787949518490336 ) ) ;
#42362=CARTESIAN_POINT ( 'NONE',  ( -109.7085897907247869, -276.4948309697917921, -293.7041084104981792 ) ) ;
#42363=AXIS2_PLACEMENT_3D ( 'NONE', #18452, #6135, #28385 ) ;
#42364=CARTESIAN_POINT ( 'NONE',  ( 34.21942695004410240, -276.0060889641903827, -255.3702799987047172 ) ) ;
#42365=CARTESIAN_POINT ( 'NONE',  ( 32.88398243018339429, -283.8999001097074597, -297.1637658701103533 ) ) ;
#42367=CARTESIAN_POINT ( 'NONE',  ( 31.56194128015845379, -289.8759331276331181, -301.3708325234615018 ) ) ;
#42368=CARTESIAN_POINT ( 'NONE',  ( -31.72090765526752065, -290.1228095979524255, -195.5214087712234345 ) ) ;
#42370=CARTESIAN_POINT ( 'NONE',  ( -27.20570452537729622, -272.8683533986801422, -197.5190438051477031 ) ) ;
#42371=CARTESIAN_POINT ( 'NONE',  ( 36.05564652922612368, -291.8403350076195011, -281.8166089304377238 ) ) ;
#42372=CARTESIAN_POINT ( 'NONE',  ( 185.7741171649701926, 251.7621132184994508, -165.9827577097485118 ) ) ;
#42374=CARTESIAN_POINT ( 'NONE',  ( -77.78549515300409212, -288.0643079586167801, -335.1298514573048237 ) ) ;
#42375=CARTESIAN_POINT ( 'NONE',  ( -108.1538423715957578, -285.8797177728571342, -291.1927510768438196 ) ) ;
#42376=CARTESIAN_POINT ( 'NONE',  ( 35.72316052809414089, -285.5247871268720701, -249.3054454384577241 ) ) ;
#42377=CARTESIAN_POINT ( 'NONE',  ( -100.9009958447769293, -285.4724550515371675, -307.4500765017594972 ) ) ;
#42378=CARTESIAN_POINT ( 'NONE',  ( -45.64766972519907284, -283.9628114373571179, -343.1006869732456153 ) ) ;
#42379=CARTESIAN_POINT ( 'NONE',  ( -97.06056401540871548, -293.1588555032605541, -224.3830303256112302 ) ) ;
#42380=CARTESIAN_POINT ( 'NONE',  ( 5.042938605749641034, -274.5638675266405357, -332.9139484170273136 ) ) ;
#42381=CARTESIAN_POINT ( 'NONE',  ( -2.570892734687665548, -274.8325777617924928, -201.6679277018994583 ) ) ;
#42382=CARTESIAN_POINT ( 'NONE',  ( -98.84446049999326078, -289.2245012691943202, -226.4666460520591045 ) ) ;
#42383=CARTESIAN_POINT ( 'NONE',  ( -31.45026642415595219, -276.9798372843007428, -347.1880273555456142 ) ) ;
#42384=CARTESIAN_POINT ( 'NONE',  ( -20.45203625092333866, -296.8142157503624503, -343.1233143870522326 ) ) ;
#42387=CARTESIAN_POINT ( 'NONE',  ( -86.04048163229326462, -284.0454562775648810, -215.2506559664484200 ) ) ;
#42388=CARTESIAN_POINT ( 'NONE',  ( 9.591820881458989589, -278.6971356682384453, -211.7945740586631871 ) ) ;
#42390=CARTESIAN_POINT ( 'NONE',  ( 29.92970205765440284, -297.2809173091810635, -194.1790562426981239 ) ) ;
#42391=CARTESIAN_POINT ( 'NONE',  ( -8.706383249097893184, -276.0158887314272533, -337.6347060179286927 ) ) ;
#42392=CARTESIAN_POINT ( 'NONE',  ( -23.36857653014567049, -296.3905295839335281, -342.7696901447928894 ) ) ;
#42393=CARTESIAN_POINT ( 'NONE',  ( 21.74139317677540006, -279.8125819635281459, -221.4665314059629964 ) ) ;
#42394=CARTESIAN_POINT ( 'NONE',  ( -7.882696117460126217, -295.5976935185100274, -337.4237935270852518 ) ) ;
#42396=CARTESIAN_POINT ( 'NONE',  ( -71.83660135248504730, -296.8137152771133174, -338.6502098201679587 ) ) ;
#42397=CARTESIAN_POINT ( 'NONE',  ( -47.27064680046883183, -297.7559347124358169, -197.9882923834420865 ) ) ;
#42398=CARTESIAN_POINT ( 'NONE',  ( -108.9177393926346582, -292.8417942542102423, -247.9153236157475533 ) ) ;
#42399=CARTESIAN_POINT ( 'NONE',  ( -102.5196037710115320, -285.2556876483272958, -229.3630585015199870 ) ) ;
#42400=CARTESIAN_POINT ( 'NONE',  ( -52.27854330543111416, -272.0025896527199620, -196.0297226417642662 ) ) ;
#42401=CARTESIAN_POINT ( 'NONE',  ( 38.29058305408145202, -287.2047751234372299, -255.9126666753702182 ) ) ;
#42402=CARTESIAN_POINT ( 'NONE',  ( -93.46133121964680868, -281.2191930362118342, -221.1234393951787069 ) ) ;
#42404=CARTESIAN_POINT ( 'NONE',  ( -41.32377650584606954, -285.0595677206560481, -197.2216244785268771 ) ) ;
#42405=CARTESIAN_POINT ( 'NONE',  ( -79.43963163530425220, -287.6200394192532599, -332.4945149792881125 ) ) ;
#42406=CARTESIAN_POINT ( 'NONE',  ( 197.9739649220119588, 291.4634315377682583, -67.91333382494548232 ) ) ;
#42407=CARTESIAN_POINT ( 'NONE',  ( 35.33625001697656387, -286.9612525715483002, -262.8842199427909918 ) ) ;
#42408=CARTESIAN_POINT ( 'NONE',  ( 13.53384431242066555, -283.3017363432580282, -327.9166570225073087 ) ) ;
#42409=CARTESIAN_POINT ( 'NONE',  ( -42.02758827201233771, -291.0531947517390563, -193.7395631467328485 ) ) ;
#42410=CARTESIAN_POINT ( 'NONE',  ( -61.81023454774331327, -281.3396145714237377, -198.1408521450441640 ) ) ;
#42411=CARTESIAN_POINT ( 'NONE',  ( -113.7195135901158949, -279.9232309594380581, -265.9195098998526419 ) ) ;
#42412=CARTESIAN_POINT ( 'NONE',  ( 26.45986893634234605, -280.9004665539023335, -234.8877506571367917 ) ) ;
#42413=CARTESIAN_POINT ( 'NONE',  ( 37.34799268838678898, -277.6398253032924117, -277.1765735041109906 ) ) ;
#42414=CARTESIAN_POINT ( 'NONE',  ( -16.50687936599918970, -294.7902771600710707, -344.5440125573325645 ) ) ;
#42415=CARTESIAN_POINT ( 'NONE',  ( -20.78857403068984055, -286.8587213615697920, -343.1473860278132406 ) ) ;
#42416=CARTESIAN_POINT ( 'NONE',  ( -107.7524451484439254, -295.7412925800470589, -249.9514864393960920 ) ) ;
#42418=ORIENTED_EDGE ( 'NONE', *, *, #27281, .T. ) ;
#42419=CARTESIAN_POINT ( 'NONE',  ( -7.902694791021886545, -284.5835498985225058, -338.7325971581332169 ) ) ;
#42420=CARTESIAN_POINT ( 'NONE',  ( -94.79270246972060932, -295.5834966995126933, -315.4329475085029912 ) ) ;
#42421=CARTESIAN_POINT ( 'NONE',  ( 38.54397403782432008, -294.4881709102701279, -258.9211454097292631 ) ) ;
#42422=CARTESIAN_POINT ( 'NONE',  ( -80.67990542881109661, -284.3087377346972744, -329.2942258662741324 ) ) ;
#42423=CARTESIAN_POINT ( 'NONE',  ( -7.770104050997200140, -273.4889504037163306, -199.4644398280292421 ) ) ;
#42424=CARTESIAN_POINT ( 'NONE',  ( -80.47656587688828722, -290.2711861293694824, -334.0862302019627350 ) ) ;
#42425=CARTESIAN_POINT ( 'NONE',  ( -34.54861462927985372, -281.1569840664961930, -346.0744203545301616 ) ) ;
#42427=CARTESIAN_POINT ( 'NONE',  ( -101.6686282695899024, -291.4424893707802653, -227.9831831999890710 ) ) ;
#42428=CARTESIAN_POINT ( 'NONE',  ( 34.78077425787379440, -288.0371026675803705, -281.8616965868361603 ) ) ;
#42431=CARTESIAN_POINT ( 'NONE',  ( 25.57469608755605961, -24.14966140349115875, -341.3741087935360383 ) ) ;
#42433=CARTESIAN_POINT ( 'NONE',  ( -4.829096099716524648, -286.1237833571632905, -337.9475929042657754 ) ) ;
#42435=CARTESIAN_POINT ( 'NONE',  ( -4.195556142615309625, -279.4200995118495712, -204.9594066443358713 ) ) ;
#42436=CARTESIAN_POINT ( 'NONE',  ( -32.67964170847187688, -273.7760883626745567, -193.5104183097055852 ) ) ;
#42437=CARTESIAN_POINT ( 'NONE',  ( -98.36633488680406856, -279.9620341449951297, -313.6964367216176583 ) ) ;
#42438=CARTESIAN_POINT ( 'NONE',  ( 203.1614497710260707, 290.3320369869807109, -82.66081499759458495 ) ) ;
#42439=CARTESIAN_POINT ( 'NONE',  ( 36.97104023705923481, -280.3516544767687719, -288.1995297295993623 ) ) ;
#42440=CARTESIAN_POINT ( 'NONE',  ( 8.791148951116039001, -280.4366319136524339, -329.1093686124274313 ) ) ;
#42441=CARTESIAN_POINT ( 'NONE',  ( -110.6505008171513538, -298.5682850794868273, -250.1716295355531656 ) ) ;
#42442=CARTESIAN_POINT ( 'NONE',  ( 34.89978769456786267, -294.1927184156310773, -281.6062306115200613 ) ) ;
#42444=CARTESIAN_POINT ( 'NONE',  ( -79.80206140066704279, -290.1497094277491442, -210.3124076780740381 ) ) ;
#42445=CARTESIAN_POINT ( 'NONE',  ( 19.95436720214620507, -275.5063312634803196, -218.9947344057348744 ) ) ;
#42446=CARTESIAN_POINT ( 'NONE',  ( -83.19058505835093342, -273.4036441152288148, -213.5554866538713270 ) ) ;
#42451=CARTESIAN_POINT ( 'NONE',  ( -66.20401008319879566, -280.7449299340070183, -202.9590445077823802 ) ) ;
#42452=CARTESIAN_POINT ( 'NONE',  ( -4.121137745965621768, -282.2442633692047025, -202.0067007805730555 ) ) ;
#42453=CARTESIAN_POINT ( 'NONE',  ( -108.9526602651009455, -283.4084199611544364, -285.7595257860030529 ) ) ;
#42454=CARTESIAN_POINT ( 'NONE',  ( -11.33220374933405239, -282.2549389893032412, -200.7771188105159865 ) ) ;
#42455=CARTESIAN_POINT ( 'NONE',  ( 36.33648845465727817, -274.0124985707211067, -268.8670370939927921 ) ) ;
#42460=CARTESIAN_POINT ( 'NONE',  ( -48.46049489216986217, -277.9929427585155395, -346.4447032779111737 ) ) ;
#42464=CARTESIAN_POINT ( 'NONE',  ( -38.67755565546019625, -285.0487173313849212, -345.7044806404859969 ) ) ;
#42465=CARTESIAN_POINT ( 'NONE',  ( 35.78304895597343460, -292.7188047607918975, -268.0431883363229417 ) ) ;
#42466=CARTESIAN_POINT ( 'NONE',  ( -4.384282607917082686, -287.9777280974648761, -339.8530659658521245 ) ) ;
#42467=CARTESIAN_POINT ( 'NONE',  ( -108.3204279705254294, -283.0678573580605644, -249.2075155727910385 ) ) ;
#42468=CARTESIAN_POINT ( 'NONE',  ( -49.50115984828789806, -284.4689485472754313, -197.7315063751577497 ) ) ;
#42469=CARTESIAN_POINT ( 'NONE',  ( -45.49604767983542075, -287.3967462372113459, -343.9238845749121083 ) ) ;
#42470=CARTESIAN_POINT ( 'NONE',  ( 5.838006246322387405, -283.6569663060549260, -329.7129794628483523 ) ) ;
#42471=CARTESIAN_POINT ( 'NONE',  ( 20.32972382687431789, -272.8899438423821948, -222.4131512750598461 ) ) ;
#42472=CARTESIAN_POINT ( 'NONE',  ( -112.3531629457156384, -282.7789410388660372, -284.0572552147507395 ) ) ;
#42473=CARTESIAN_POINT ( 'NONE',  ( -95.83128075245272726, -297.9062562714833575, -317.3278898714050342 ) ) ;
#42474=CARTESIAN_POINT ( 'NONE',  ( -31.01222614726124860, -284.1317716816291181, -195.4484320985835382 ) ) ;
#42475=CARTESIAN_POINT ( 'NONE',  ( -92.39320718732552962, -280.1807206404401995, -222.0435897916533463 ) ) ;
#42476=CARTESIAN_POINT ( 'NONE',  ( 8.667988948866881316, -288.6812277524787191, -210.9209216966050917 ) ) ;
#42479=CARTESIAN_POINT ( 'NONE',  ( 36.94609038373248922, -295.6491640990642509, -284.2383344620357661 ) ) ;
#42480=CARTESIAN_POINT ( 'NONE',  ( -100.8827153437524657, -276.0153548599132023, -310.3021231736551613 ) ) ;
#42481=CARTESIAN_POINT ( 'NONE',  ( -109.3189808297879750, -290.0919167419311862, -243.3128910110611116 ) ) ;
#42482=CARTESIAN_POINT ( 'NONE',  ( -10.21469398820136831, -293.0919215033308092, -338.9946808617684724 ) ) ;
#42483=CARTESIAN_POINT ( 'NONE',  ( -104.8887827829167065, -277.6233996011955583, -241.4019207983978106 ) ) ;
#42484=CARTESIAN_POINT ( 'NONE',  ( -97.42953907880669817, -271.2364393961005931, -226.3350328184559999 ) ) ;
#42485=CARTESIAN_POINT ( 'NONE',  ( -106.1784018442980937, -292.2101778352040355, -244.4726537207301931 ) ) ;
#42486=CARTESIAN_POINT ( 'NONE',  ( -4.771743288812468897, -285.1233781216987495, -337.9199732462171255 ) ) ;
#42487=CARTESIAN_POINT ( 'NONE',  ( -14.01258554482040708, -293.2347395927417324, -343.0141300620367133 ) ) ;
#42488=CARTESIAN_POINT ( 'NONE',  ( -94.71348264742380252, -291.5027692296777104, -316.7822229693273357 ) ) ;
#42489=CARTESIAN_POINT ( 'NONE',  ( 35.32457609781123864, -291.5093369746655867, -248.1443154795454120 ) ) ;
#42490=CARTESIAN_POINT ( 'NONE',  ( -102.9430045682343433, -292.4279951046752331, -236.9039410442110523 ) ) ;
#42492=CARTESIAN_POINT ( 'NONE',  ( -18.42190869602884362, -289.6050660920769815, -341.0866118805447513 ) ) ;
#42494=CARTESIAN_POINT ( 'NONE',  ( -113.9926312953178353, -291.7461829576876653, -271.2395999151335673 ) ) ;
#42495=CARTESIAN_POINT ( 'NONE',  ( 38.06466923558203774, -279.5671901812859232, -269.9646359496893524 ) ) ;
#42496=CARTESIAN_POINT ( 'NONE',  ( -12.26020631080762868, -292.3876102128842263, -201.7512875080602157 ) ) ;
#42497=CARTESIAN_POINT ( 'NONE',  ( -2.390141635068330661, -280.5016501009009176, -201.7359788623843428 ) ) ;
#42499=CARTESIAN_POINT ( 'NONE',  ( 24.23563647454788494, -281.8338757631203748, -316.5560950745872333 ) ) ;
#42500=CARTESIAN_POINT ( 'NONE',  ( 28.12527861860371914, -285.0635795148411944, -233.6614189914476469 ) ) ;
#42501=CARTESIAN_POINT ( 'NONE',  ( 31.17042443314550937, -279.3147150633383831, -241.7787061532553423 ) ) ;
#42502=CARTESIAN_POINT ( 'NONE',  ( -109.7826122830774551, -282.8039599091048331, -250.7415842636285390 ) ) ;
#42504=CARTESIAN_POINT ( 'NONE',  ( -64.47750154657505561, -278.1843143148682316, -198.9867079554612985 ) ) ;
#42505=CARTESIAN_POINT ( 'NONE',  ( -75.93920986785983018, -284.4700130524016686, -204.0298806287281934 ) ) ;
#42506=CARTESIAN_POINT ( 'NONE',  ( -32.69095757330136109, -274.9150655198245659, -197.3350561345241658 ) ) ;
#42508=CARTESIAN_POINT ( 'NONE',  ( 34.72666839505038183, -294.9441368203573006, -254.4096540843970899 ) ) ;
#42509=CARTESIAN_POINT ( 'NONE',  ( -36.96103440260684891, -275.4821281253670122, -193.9383408897356276 ) ) ;
#42510=CARTESIAN_POINT ( 'NONE',  ( -97.66868864158274732, -277.6466347378795945, -311.5040632305970689 ) ) ;
#42511=CARTESIAN_POINT ( 'NONE',  ( -106.5125782799321001, -290.2830593939783057, -304.3111369788155685 ) ) ;
#42512=CARTESIAN_POINT ( 'NONE',  ( -4.265463125965251123, -278.5645641888096407, -202.4110404023321905 ) ) ;
#42513=CARTESIAN_POINT ( 'NONE',  ( 17.49109674441720585, -292.6423632383825293, -216.2271383537219265 ) ) ;
#42515=CARTESIAN_POINT ( 'NONE',  ( -103.7647076125308843, -290.0259248478650420, -239.5164665159246056 ) ) ;
#42516=CARTESIAN_POINT ( 'NONE',  ( 19.82621375535443065, -292.2238954035275924, -318.9083143378635441 ) ) ;
#42519=CARTESIAN_POINT ( 'NONE',  ( -65.34475253577710419, -291.1836363983406386, -202.8656139963957230 ) ) ;
#42520=CARTESIAN_POINT ( 'NONE',  ( 30.91033621190086578, -278.8380690714489560, -254.8156830097664738 ) ) ;
#42521=CARTESIAN_POINT ( 'NONE',  ( -110.1264353503709401, -295.3027528842199558, -294.7578909529135558 ) ) ;
#42522=CARTESIAN_POINT ( 'NONE',  ( -81.26465132796487012, -284.9503086261767066, -333.0679782429864417 ) ) ;
#42523=CARTESIAN_POINT ( 'NONE',  ( -2.184521322503762519, -286.3642642267885208, -206.3280554522691830 ) ) ;
#42524=CARTESIAN_POINT ( 'NONE',  ( 12.22825554471529408, -277.8678339576953249, -324.9604371279157249 ) ) ;
#42525=CARTESIAN_POINT ( 'NONE',  ( -74.13461051777825617, -293.5638124406008274, -335.3082391557379083 ) ) ;
#42526=CARTESIAN_POINT ( 'NONE',  ( -95.55677961956858724, -297.6765801856430471, -316.0664627061902934 ) ) ;
#42528=CARTESIAN_POINT ( 'NONE',  ( 22.78232720893039698, -274.9320457407357594, -312.5462334195946710 ) ) ;
#42531=CARTESIAN_POINT ( 'NONE',  ( -109.8295243780542876, -296.5460091089748857, -244.4524393790357237 ) ) ;
#42532=CARTESIAN_POINT ( 'NONE',  ( 13.15015081751855597, -290.2605204887556738, -325.1293301925349510 ) ) ;
#42534=CARTESIAN_POINT ( 'NONE',  ( 21.26016509809543109, -288.8161046337660878, -314.0823504299175966 ) ) ;
#42536=CARTESIAN_POINT ( 'NONE',  ( -14.28696721684780080, -279.4026026725536553, -197.0844904720465536 ) ) ;
#42537=CARTESIAN_POINT ( 'NONE',  ( -13.80534638719844942, -295.4059249580225810, -343.5687189468729343 ) ) ;
#42538=CARTESIAN_POINT ( 'NONE',  ( -73.85319858481622646, -287.6712070385224251, -336.7627981140441875 ) ) ;
#42539=CARTESIAN_POINT ( 'NONE',  ( -104.5823670025761913, -296.3982141380537314, -307.9458956226947635 ) ) ;
#42540=CARTESIAN_POINT ( 'NONE',  ( 32.36825079043457976, -294.1734330795222832, -292.1007184785422055 ) ) ;
#42544=CARTESIAN_POINT ( 'NONE',  ( -57.09260349216318531, -290.8224297304331571, -344.1219610217855802 ) ) ;
#42545=CARTESIAN_POINT ( 'NONE',  ( -55.56934967048407970, -295.3380690714490129, -190.3538533559490702 ) ) ;
#42547=CARTESIAN_POINT ( 'NONE',  ( -38.16048880506484409, -279.3907338161644134, -193.4674097080047375 ) ) ;
#42548=CARTESIAN_POINT ( 'NONE',  ( -71.01769606448635841, -285.4976827002761297, -337.2032521700472785 ) ) ;
#42549=CARTESIAN_POINT ( 'NONE',  ( -32.32682456429676421, -284.6889262500657196, -194.1020210459960254 ) ) ;
#42550=CARTESIAN_POINT ( 'NONE',  ( 20.61961945506797633, -286.2796624455659753, -317.0708560901406372 ) ) ;
#42551=CARTESIAN_POINT ( 'NONE',  ( -23.14671025493263556, -278.7330267318222923, -344.8376029907565226 ) ) ;
#42553=CARTESIAN_POINT ( 'NONE',  ( -76.35581941721268606, -277.5894237337617483, -332.1206373169924859 ) ) ;
#42554=CARTESIAN_POINT ( 'NONE',  ( -92.27956894233068397, -278.5883127697608188, -222.1163255152069667 ) ) ;
#42555=CARTESIAN_POINT ( 'NONE',  ( 24.22347928239249271, -276.0213114192907256, -224.6312459652183406 ) ) ;
#42556=CARTESIAN_POINT ( 'NONE',  ( -90.77016909999454697, -278.1099401161383184, -215.3926723503662970 ) ) ;
#42557=CARTESIAN_POINT ( 'NONE',  ( 197.5292130366077856, 288.3118105299622584, -96.80481239046156361 ) ) ;
#42558=CARTESIAN_POINT ( 'NONE',  ( -87.89047171050665952, -274.3071897815528359, -212.5181075685498797 ) ) ;
#42559=CARTESIAN_POINT ( 'NONE',  ( -37.62384221459190314, -299.4739495959235569, -193.9508654540946111 ) ) ;
#42560=CARTESIAN_POINT ( 'NONE',  ( -106.6379572354042296, -286.6233781216988064, -303.7686719486574702 ) ) ;
#42561=CARTESIAN_POINT ( 'NONE',  ( 82.66356608220550584, -298.4024577471378166, -193.1360764112615982 ) ) ;
#42563=CARTESIAN_POINT ( 'NONE',  ( -10.65018257429869308, -287.4883265503664234, -202.0702413516283684 ) ) ;
#42564=CARTESIAN_POINT ( 'NONE',  ( -40.79318215999495578, -287.7695687098921553, -194.4013701814462536 ) ) ;
#42565=CARTESIAN_POINT ( 'NONE',  ( 12.21882348805063501, -287.6893672464220799, -324.1667274881333469 ) ) ;
#42566=CARTESIAN_POINT ( 'NONE',  ( -61.21853497581030012, -282.8615899978443622, -343.5565139582915890 ) ) ;
#42567=CARTESIAN_POINT ( 'NONE',  ( -39.70667593311462440, -278.4218615285074634, -196.5863614139851165 ) ) ;
#42568=CARTESIAN_POINT ( 'NONE',  ( 15.89914735725999151, -288.6769859940899323, -218.6283658915252204 ) ) ;
#42569=CARTESIAN_POINT ( 'NONE',  ( 35.72280838892917387, -279.9015233371092108, -260.3744474690736865 ) ) ;
#42571=CARTESIAN_POINT ( 'NONE',  ( 9.994378199043083555, -277.6988324975472437, -326.5797907277363947 ) ) ;
#42572=CARTESIAN_POINT ( 'NONE',  ( 25.43164424310218763, -276.5580179711071196, -307.7442114608942916 ) ) ;
#42573=CARTESIAN_POINT ( 'NONE',  ( -77.93905190224344892, -288.3793034123935399, -335.3834796541093510 ) ) ;
#42575=CARTESIAN_POINT ( 'NONE',  ( -33.05750822365979502, -283.8023386265159047, -347.0932224889459121 ) ) ;
#42576=CARTESIAN_POINT ( 'NONE',  ( -61.20662319587470535, -283.8461257744933164, -343.5603980248732796 ) ) ;
#42577=CARTESIAN_POINT ( 'NONE',  ( 11.30424099245688652, -280.9157324153339346, -215.9316000994883495 ) ) ;
#42579=EDGE_LOOP ( 'NONE', ( #23946, #24064, #39386, #44636 ) ) ;
#42581=CARTESIAN_POINT ( 'NONE',  ( -86.56368792329394068, -291.5875671768767461, -328.0277636718988106 ) ) ;
#42582=CARTESIAN_POINT ( 'NONE',  ( -67.87256616255660902, -288.1294418634895464, -340.5121300422136983 ) ) ;
#42583=CARTESIAN_POINT ( 'NONE',  ( -99.47378243058825831, -272.1442836178328548, -231.5924089939479984 ) ) ;
#42584=CARTESIAN_POINT ( 'NONE',  ( 37.66372760493411675, -292.6877388643204654, -253.3462670035110875 ) ) ;
#42585=CARTESIAN_POINT ( 'NONE',  ( -64.09044247684056472, -287.8872571468643855, -339.0832292362473481 ) ) ;
#42586=CARTESIAN_POINT ( 'NONE',  ( 34.75752506226930194, -292.0102569731087101, -287.1403857160945563 ) ) ;
#42587=CARTESIAN_POINT ( 'NONE',  ( 34.67673903866996454, -288.9438535386589706, -284.5850729517826494 ) ) ;
#42588=CARTESIAN_POINT ( 'NONE',  ( 31.98288692825981272, -296.4805209788415823, -303.7098442033569654 ) ) ;
#42589=CARTESIAN_POINT ( 'NONE',  ( 9.012370294954282102, -290.4166657428516487, -329.3873684085881450 ) ) ;
#42590=CARTESIAN_POINT ( 'NONE',  ( -112.5559253764166812, -288.5414624975909419, -271.1826781763828649 ) ) ;
#42591=CARTESIAN_POINT ( 'NONE',  ( -48.27292950850284114, -293.9133395085021334, -196.1101237109748467 ) ) ;
#42592=CARTESIAN_POINT ( 'NONE',  ( -93.59513383851965784, -284.8301283410953033, -317.2541840434030860 ) ) ;
#42593=CARTESIAN_POINT ( 'NONE',  ( -33.65537278147974831, -294.0986121196559111, -195.2848939226211940 ) ) ;
#42594=CARTESIAN_POINT ( 'NONE',  ( -114.1561780732172480, -273.4200912208958130, -270.3721689257164940 ) ) ;
#42596=CARTESIAN_POINT ( 'NONE',  ( -66.91389818336824646, -275.6464130736508764, -201.0510039518020449 ) ) ;
#42597=CARTESIAN_POINT ( 'NONE',  ( -32.14441068128075329, -282.1820803459872877, -343.3377574606344638 ) ) ;
#42598=CARTESIAN_POINT ( 'NONE',  ( -0.2854021067749158425, -280.5591494292785342, -335.5671869221244492 ) ) ;
#42599=CARTESIAN_POINT ( 'NONE',  ( -88.50554834642690594, -294.9449912121329476, -327.7597775610984172 ) ) ;
#42600=CARTESIAN_POINT ( 'NONE',  ( 34.82678483088223231, -273.5776771163112926, -253.8823245216564999 ) ) ;
#42601=CARTESIAN_POINT ( 'NONE',  ( -111.3960647627474003, -276.7362591262742626, -262.3012767681219657 ) ) ;
#42602=CARTESIAN_POINT ( 'NONE',  ( -110.7055576525951039, -297.9244301265383683, -266.0036088324801540 ) ) ;
#42603=CARTESIAN_POINT ( 'NONE',  ( 30.73363665616459883, -273.6765033344636322, -235.6573024427248697 ) ) ;
#42604=CARTESIAN_POINT ( 'NONE',  ( -67.52038575554564659, -296.8812532099888131, -337.4914125938276470 ) ) ;
#42605=DIRECTION ( 'NONE',  ( 0.000000000000000000, 0.000000000000000000, 1.000000000000000000 ) ) ;
#42606=CARTESIAN_POINT ( 'NONE',  ( -96.53304938826724424, -296.7542684128148949, -313.3823332750778263 ) ) ;
#42607=DIRECTION ( 'NONE',  ( -1.000000000000000000, -0.000000000000000000, -0.000000000000000000 ) ) ;
#42608=CARTESIAN_POINT ( 'NONE',  ( 24.21634886488942939, -284.9843362706011476, -226.8760791316890959 ) ) ;
#42609=CARTESIAN_POINT ( 'NONE',  ( -37.82251735037001339, -298.0459637686756764, -197.3627014600165239 ) ) ;
#42610=CARTESIAN_POINT ( 'NONE',  ( -9.993960832771835001, -286.3994108159059806, -198.3244508398656478 ) ) ;
#42611=CARTESIAN_POINT ( 'NONE',  ( 7.918650267466007087, -288.1195259727757048, -332.6943760447730369 ) ) ;
#42612=CARTESIAN_POINT ( 'NONE',  ( -112.7201997012685837, -298.5053538625817851, -272.4499071714736829 ) ) ;
#42613=CARTESIAN_POINT ( 'NONE',  ( 37.54242783184480459, -291.5575744174519741, -270.7953604001459098 ) ) ;
#42614=CARTESIAN_POINT ( 'NONE',  ( -33.91222804012959813, -279.2914393933908173, -193.5991642423914811 ) ) ;
#42615=CARTESIAN_POINT ( 'NONE',  ( 31.95455697924147387, -291.4809262143061801, -303.7686719486574134 ) ) ;
#42616=DIRECTION ( 'NONE',  ( 0.000000000000000000, 0.000000000000000000, 1.000000000000000000 ) ) ;
#42617=CARTESIAN_POINT ( 'NONE',  ( -1.981687420488145390, -285.3260362426477741, -205.9861276708301148 ) ) ;
#42619=CARTESIAN_POINT ( 'NONE',  ( -103.4168970293110306, -288.0797640049244137, -305.9546600654516055 ) ) ;
#42620=CARTESIAN_POINT ( 'NONE',  ( -37.84823625288498761, -299.6458330807033121, -196.5628535124512268 ) ) ;
#42621=CARTESIAN_POINT ( 'NONE',  ( -3.931759451526023241, -281.9094486853182389, -201.6271221130625690 ) ) ;
#42622=CARTESIAN_POINT ( 'NONE',  ( -92.44245509465827126, -295.2890533444373773, -218.8815948689192794 ) ) ;
#42623=CARTESIAN_POINT ( 'NONE',  ( 9.908696275385604935, -282.3801926386418018, -326.0728993574523997 ) ) ;
#42624=CARTESIAN_POINT ( 'NONE',  ( -91.63703121313025690, -297.4708200152910536, -215.7624272760778581 ) ) ;
#42625=CARTESIAN_POINT ( 'NONE',  ( -33.78935643706599024, -299.6175343049769140, -196.6668402802768014 ) ) ;
#42626=CARTESIAN_POINT ( 'NONE',  ( 37.70894528338921958, -283.5466024423273552, -269.9160369944169702 ) ) ;
#42627=CARTESIAN_POINT ( 'NONE',  ( -110.3348058049926266, -295.5247977681781890, -276.9087912148806936 ) ) ;
#42632=CARTESIAN_POINT ( 'NONE',  ( -65.92267374842099059, -285.4078138589302966, -339.3313455811912149 ) ) ;
#42633=CARTESIAN_POINT ( 'NONE',  ( 104.1717476309105166, -299.5541904835127980, -197.7570935515975350 ) ) ;
#42634=CARTESIAN_POINT ( 'NONE',  ( 35.77081079830085031, -291.2666405000204577, -287.0812184334320705 ) ) ;
#42635=CARTESIAN_POINT ( 'NONE',  ( 37.48002216566043643, -274.5294865096090575, -252.8147467647210931 ) ) ;
#42636=CARTESIAN_POINT ( 'NONE',  ( -34.85515696084014081, -291.9175750985450009, -197.4034788513308456 ) ) ;
#42638=CARTESIAN_POINT ( 'NONE',  ( 9.704430016058637420, -282.2331093358340013, -213.5727527777936245 ) ) ;
#42639=CARTESIAN_POINT ( 'NONE',  ( -7.162059756873111915, -278.2496160505488092, -337.7082019881324868 ) ) ;
#42640=CARTESIAN_POINT ( 'NONE',  ( -106.4648393807225233, -285.5570400589816700, -302.9279402276478095 ) ) ;
#42641=CARTESIAN_POINT ( 'NONE',  ( 24.02290014644300342, -279.7907373501017787, -230.0013787271210504 ) ) ;
#42642=CARTESIAN_POINT ( 'NONE',  ( -99.28672050622678569, -279.9796998016676639, -312.6436805779548536 ) ) ;
#42643=CARTESIAN_POINT ( 'NONE',  ( -37.60766213542171954, -298.0489080631367074, -193.3615773072374679 ) ) ;
#42644=CARTESIAN_POINT ( 'NONE',  ( 10.52439761362969683, -276.2454253879897124, -330.7436833701567025 ) ) ;
#42645=CARTESIAN_POINT ( 'NONE',  ( 27.47663568408251322, -294.9796954283365835, -233.6513186969969809 ) ) ;
#42648=CARTESIAN_POINT ( 'NONE',  ( -100.6100759521699501, -294.1336626216511831, -312.1383907948717820 ) ) ;
#42649=CARTESIAN_POINT ( 'NONE',  ( -59.48833213081312721, -273.2652893790467488, -200.6840547687569654 ) ) ;
#42650=CARTESIAN_POINT ( 'NONE',  ( 37.64031465244426045, -294.8936142852089688, -256.2046631454692829 ) ) ;
#42651=CARTESIAN_POINT ( 'NONE',  ( 27.77651910220412290, -295.2886875565050673, -310.8046546133618904 ) ) ;
#42652=CARTESIAN_POINT ( 'NONE',  ( -69.52389536483657650, -291.4768901203700011, -337.9209784098173941 ) ) ;
#42654=CARTESIAN_POINT ( 'NONE',  ( -65.03470287340681466, -275.4144774329361667, -339.9368454969134064 ) ) ;
#42655=CARTESIAN_POINT ( 'NONE',  ( 18.53195299637424753, -278.1612296395080648, -319.5682515581325447 ) ) ;
#42656=CARTESIAN_POINT ( 'NONE',  ( -53.48502648492690525, -293.3405400750720560, -343.0826061733354777 ) ) ;
#42657=CARTESIAN_POINT ( 'NONE',  ( 38.17857347994645068, -283.3352610884610385, -264.2788689955200994 ) ) ;
#42658=CARTESIAN_POINT ( 'NONE',  ( -62.65676387679056347, -284.6352500180802281, -201.5074682865840430 ) ) ;
#42659=CARTESIAN_POINT ( 'NONE',  ( -105.3677979232747077, -263.0180028947901860, -317.1570552232428213 ) ) ;
#42661=CARTESIAN_POINT ( 'NONE',  ( -108.9488684060140997, -284.4074610409488173, -256.0607355377569547 ) ) ;
#42662=CARTESIAN_POINT ( 'NONE',  ( -14.33365010659369077, -281.4232006105839332, -197.1472461593778860 ) ) ;
#42663=CARTESIAN_POINT ( 'NONE',  ( -69.61151350320699294, -284.4317125872794918, -200.8726032522603475 ) ) ;
#42664=CARTESIAN_POINT ( 'NONE',  ( -112.7672430482424488, -279.6733725233076484, -256.0146379608212328 ) ) ;
#42666=CARTESIAN_POINT ( 'NONE',  ( -110.7680358687956641, -279.8096234922635404, -291.1284233754840898 ) ) ;
#42667=CARTESIAN_POINT ( 'NONE',  ( 17.36665895637873192, -273.6952119285918457, -314.0302885647153062 ) ) ;
#42668=CARTESIAN_POINT ( 'NONE',  ( 85.80530294649854284, 82.61953402769070465, -302.2778766101830001 ) ) ;
#42670=CARTESIAN_POINT ( 'NONE',  ( -39.24390427567689699, -300.0284663726370127, -195.3724915477045556 ) ) ;
#42671=CARTESIAN_POINT ( 'NONE',  ( -11.14275193769495864, -278.4152501914209097, -200.4103682797326371 ) ) ;
#42672=CARTESIAN_POINT ( 'NONE',  ( -113.1779438795799138, -292.3728570457565183, -265.5821907631614067 ) ) ;
#42673=CARTESIAN_POINT ( 'NONE',  ( -5.504603325692409399, -293.9705048623722519, -336.1799006659069846 ) ) ;
#42674=CARTESIAN_POINT ( 'NONE',  ( -114.0516562745819158, -289.9774362787086375, -276.9420829750088160 ) ) ;
#42676=CARTESIAN_POINT ( 'NONE',  ( 32.86793026969274223, -292.5154332909403365, -300.6478447484029175 ) ) ;
#42677=CARTESIAN_POINT ( 'NONE',  ( -22.27683532998981519, -284.6480234467157970, -198.0626258528485266 ) ) ;
#42678=CARTESIAN_POINT ( 'NONE',  ( -37.57725767459377408, -293.9096242184923540, -196.1136340414212782 ) ) ;
#42679=CARTESIAN_POINT ( 'NONE',  ( -56.43096508852794813, -284.6185460907389029, -341.3318403965304242 ) ) ;
#42681=CARTESIAN_POINT ( 'NONE',  ( -112.9423837617850381, -291.6604651000007493, -257.0435788917860123 ) ) ;
#42682=CARTESIAN_POINT ( 'NONE',  ( -22.18775952995407863, -280.7437398214368613, -198.8365200227580942 ) ) ;
#42683=CARTESIAN_POINT ( 'NONE',  ( 38.21208988301704323, -292.5069109098688500, -283.0751192075867948 ) ) ;
#42684=CARTESIAN_POINT ( 'NONE',  ( -14.98943083880696037, -289.5727613191414207, -343.9322963618342897 ) ) ;
#42685=CARTESIAN_POINT ( 'NONE',  ( -98.97607301728342577, -290.4310792291598773, -316.4342972827571430 ) ) ;
#42686=CARTESIAN_POINT ( 'NONE',  ( 15.97301630148994001, -287.0012732660467236, -220.4774434567572712 ) ) ;
#42689=CARTESIAN_POINT ( 'NONE',  ( 35.19415262035013825, -295.6937470927641129, -292.4217990055070686 ) ) ;
#42690=CARTESIAN_POINT ( 'NONE',  ( -104.8107636197279646, -295.7074362789515476, -234.1763010823696618 ) ) ;
#42692=CARTESIAN_POINT ( 'NONE',  ( -105.7297198731176451, -277.9613814299054866, -244.0182391773769837 ) ) ;
#42693=CARTESIAN_POINT ( 'NONE',  ( -35.51895491348318501, -273.5820732781861579, -193.4311308773412463 ) ) ;
#42694=CARTESIAN_POINT ( 'NONE',  ( -47.91143771770327220, -293.6687457674160555, -343.3442817792142137 ) ) ;
#42695=CARTESIAN_POINT ( 'NONE',  ( 10.33365654855795945, -278.1437280896068955, -326.9741410137662569 ) ) ;
#42696=CARTESIAN_POINT ( 'NONE',  ( -94.71821571352488434, -271.3481332440125016, -223.2370987455944373 ) ) ;
#42698=CARTESIAN_POINT ( 'NONE',  ( 36.03958236762688472, -294.7982955396258262, -273.4906789686825732 ) ) ;
#42699=CARTESIAN_POINT ( 'NONE',  ( -31.56433566922716594, -296.0573199253470875, -343.4925497855322760 ) ) ;
#42702=CARTESIAN_POINT ( 'NONE',  ( -96.76848585895108101, -295.1817193915935036, -224.3133459985474758 ) ) ;
#42703=CARTESIAN_POINT ( 'NONE',  ( -23.39113940076908094, -298.8739271444148358, -193.4615530850009577 ) ) ;
#42704=CARTESIAN_POINT ( 'NONE',  ( -53.55587437105933191, -287.8389979442837898, -342.1418637924992368 ) ) ;
#42705=CARTESIAN_POINT ( 'NONE',  ( -107.2905268654574229, -274.9058821284872351, -243.1592330861918470 ) ) ;
#42706=CARTESIAN_POINT ( 'NONE',  ( -110.0457636035864653, -273.3621037239402654, -245.1887907697699518 ) ) ;
#42708=CARTESIAN_POINT ( 'NONE',  ( -104.9798918036931781, -296.5169415369581998, -297.8777041362385489 ) ) ;
#42710=CARTESIAN_POINT ( 'NONE',  ( -111.6195576906492448, -280.6942984741440341, -257.6643987142851984 ) ) ;
#42711=CARTESIAN_POINT ( 'NONE',  ( -25.45558560918054880, -278.8854412896631629, -194.7832207286726316 ) ) ;
#42712=CARTESIAN_POINT ( 'NONE',  ( -38.73902342481922290, -282.4178376508589281, -347.2464889879695420 ) ) ;
#42713=CARTESIAN_POINT ( 'NONE',  ( 27.55833933201302699, -275.4431730433088887, -311.7068714345336389 ) ) ;
#42714=CARTESIAN_POINT ( 'NONE',  ( 14.63074538973157424, -279.1687439922761769, -214.5637026863836638 ) ) ;
#42715=CARTESIAN_POINT ( 'NONE',  ( -38.12463413549750868, -278.0422048580156797, -195.1985245915314522 ) ) ;
#42716=CARTESIAN_POINT ( 'NONE',  ( -11.26457354804663069, -272.9733113944863021, -201.4926895191075289 ) ) ;
#42717=CARTESIAN_POINT ( 'NONE',  ( 25.37001462644079197, -278.1084698181304589, -311.5902184319775756 ) ) ;
#42719=CARTESIAN_POINT ( 'NONE',  ( -58.45319697019549920, -289.8006491648515066, -198.0236346052819840 ) ) ;
#42720=CARTESIAN_POINT ( 'NONE',  ( -98.34826317967218756, -291.1792842460076258, -223.3589437731529870 ) ) ;
#42721=CARTESIAN_POINT ( 'NONE',  ( -9.857859013599144404, -278.6941960407934289, -340.3230140734858082 ) ) ;
#42722=CARTESIAN_POINT ( 'NONE',  ( -57.37190185508347895, -271.7936214766053240, -198.0311596538433321 ) ) ;
#42725=CARTESIAN_POINT ( 'NONE',  ( -95.39336738838214558, -283.2066959169408165, -222.8543224466426693 ) ) ;
#42728=CARTESIAN_POINT ( 'NONE',  ( 26.12838274646293257, -292.8500508480920530, -307.2213822781752697 ) ) ;
#42729=CARTESIAN_POINT ( 'NONE',  ( 35.73348645255310174, -285.8613086429143095, -283.4333246870743892 ) ) ;
#42732=CARTESIAN_POINT ( 'NONE',  ( -23.16509362626534241, -292.8708136334317942, -344.0621099610601163 ) ) ;
#42733=CARTESIAN_POINT ( 'NONE',  ( -111.0464106232770831, -283.2839208396907225, -250.4061133829896164 ) ) ;
#42734=CARTESIAN_POINT ( 'NONE',  ( -67.65329937286229267, -281.2478050768619937, -203.0595653792132396 ) ) ;
#42735=CARTESIAN_POINT ( 'NONE',  ( -113.7569738163876849, -285.8334838231838262, -264.2950429750109151 ) ) ;
#42736=CARTESIAN_POINT ( 'NONE',  ( -14.51058288484636094, -278.5838453107477903, -197.8303376636982307 ) ) ;
#42737=CARTESIAN_POINT ( 'NONE',  ( 28.80995496453565607, -287.1353106951205518, -239.4910916057096699 ) ) ;
#42739=CARTESIAN_POINT ( 'NONE',  ( -59.35410140863530870, -278.7680755165813480, -340.5809805992865336 ) ) ;
#42740=CARTESIAN_POINT ( 'NONE',  ( -109.0475500006786689, -279.5469551311566647, -255.7767043200873616 ) ) ;
#42741=CARTESIAN_POINT ( 'NONE',  ( -40.76748788169187776, -287.9892841666302843, -195.0327482804862598 ) ) ;
#42743=CARTESIAN_POINT ( 'NONE',  ( -107.7721715813901255, -296.7840241410740418, -239.1077837069504426 ) ) ;
#42744=CARTESIAN_POINT ( 'NONE',  ( -64.39399362766693002, -291.3867065957127807, -339.9867694047253508 ) ) ;
#42746=CARTESIAN_POINT ( 'NONE',  ( -2.659677404128715672, -282.9805209788415823, -198.2697987213421698 ) ) ;
#42748=CARTESIAN_POINT ( 'NONE',  ( -60.28666473558980954, -271.7553288441165478, -198.7277929964787120 ) ) ;
#42749=CARTESIAN_POINT ( 'NONE',  ( 38.02228521017593721, -292.0942840304360288, -281.6176773778514644 ) ) ;
#42750=CARTESIAN_POINT ( 'NONE',  ( -84.52261865440348743, -295.2298744072514296, -326.2123975259087842 ) ) ;
#42751=CARTESIAN_POINT ( 'NONE',  ( 35.44706747601616570, -289.2237518526308691, -281.9526647420209429 ) ) ;
#42752=CARTESIAN_POINT ( 'NONE',  ( 28.67524911578215097, -282.8628173275653808, -236.7850818899946148 ) ) ;
#42753=CARTESIAN_POINT ( 'NONE',  ( -8.439059609532264972, -290.1064168208470164, -341.1088872307944939 ) ) ;
#42754=CARTESIAN_POINT ( 'NONE',  ( -91.23915194801482187, -291.1138662782858546, -324.7344563100068626 ) ) ;
#42755=CARTESIAN_POINT ( 'NONE',  ( -45.84150799167230872, -285.1599463806196582, -344.9303107361408820 ) ) ;
#42756=CARTESIAN_POINT ( 'NONE',  ( -111.8269004374234186, -278.4739295689862502, -289.9309878473421804 ) ) ;
#42757=CARTESIAN_POINT ( 'NONE',  ( 18.44959431718224963, -292.3387481116369031, -321.3945915641779720 ) ) ;
#42758=CARTESIAN_POINT ( 'NONE',  ( 30.72280569084552937, -280.9192817435474581, -234.2443416742731301 ) ) ;
#42759=CARTESIAN_POINT ( 'NONE',  ( -35.38105394294588990, -275.9374035450653082, -196.1390931051824396 ) ) ;
#42760=CARTESIAN_POINT ( 'NONE',  ( 35.78497577281001440, -296.2662352645559167, -287.0191576251351080 ) ) ;
#42761=CARTESIAN_POINT ( 'NONE',  ( 29.63910407537412794, -274.2632538661408717, -306.3545479852188009 ) ) ;
#42764=CARTESIAN_POINT ( 'NONE',  ( -1.930766155255069894, -280.0423880801637324, -206.4545127141937257 ) ) ;
#42766=CARTESIAN_POINT ( 'NONE',  ( 19.59241879461066560, -277.4566347288656516, -321.6302877564377241 ) ) ;
#42767=CARTESIAN_POINT ( 'NONE',  ( -73.14934157785657476, -298.9927627113842163, -206.0712452837533419 ) ) ;
#42768=CARTESIAN_POINT ( 'NONE',  ( -110.0058332601304301, -283.2980626186882205, -295.1147837489177732 ) ) ;
#42769=CARTESIAN_POINT ( 'NONE',  ( -85.32517614939537509, -291.4855762858202297, -326.7808552704847216 ) ) ;
#42770=CARTESIAN_POINT ( 'NONE',  ( -2.937169867794221290, -276.0992200337769304, -202.3556237322580955 ) ) ;
#42772=CARTESIAN_POINT ( 'NONE',  ( -111.9660026560661663, -274.0796304152542007, -253.4936419587741625 ) ) ;
#42775=CARTESIAN_POINT ( 'NONE',  ( 37.47595382155799371, -295.5932523172907622, -273.5421194629119555 ) ) ;
#42776=CARTESIAN_POINT ( 'NONE',  ( -29.27164136142819473, -280.9496414992527775, -344.8098152834119787 ) ) ;
#42778=CARTESIAN_POINT ( 'NONE',  ( -111.2106790195318951, -290.4906165075586841, -248.7019802093065834 ) ) ;
#42779=CARTESIAN_POINT ( 'NONE',  ( 19.54593736581788832, -274.2443485069447888, -318.6896137785293490 ) ) ;
#42780=CARTESIAN_POINT ( 'NONE',  ( 31.97572659130898387, -288.7420122456922513, -238.5871368303445479 ) ) ;
#42781=CARTESIAN_POINT ( 'NONE',  ( -65.43274500006812389, -290.5964070528142429, -202.6340391450372067 ) ) ;
#42783=CARTESIAN_POINT ( 'NONE',  ( -107.2000967268968736, -288.7273052291942577, -301.4495338470833303 ) ) ;
#42784=CARTESIAN_POINT ( 'NONE',  ( -74.98687117398149837, -291.2028263959568335, -207.7326972734991557 ) ) ;
#42786=CARTESIAN_POINT ( 'NONE',  ( 27.19215870989951611, -289.1786753810128516, -311.8942350472209455 ) ) ;
#42788=CARTESIAN_POINT ( 'NONE',  ( 20.04171244583395506, -276.5224557371282117, -315.5391065248404061 ) ) ;
#42789=CARTESIAN_POINT ( 'NONE',  ( -16.60373590580135073, -293.7107795455372639, -344.2499212861386582 ) ) ;
#42790=CARTESIAN_POINT ( 'NONE',  ( -92.35501396645300076, -284.4655315012472556, -324.0905148431945122 ) ) ;
#42792=CARTESIAN_POINT ( 'NONE',  ( -57.75441463760440541, -286.1289585621425431, -196.0827022284918542 ) ) ;
#42793=CARTESIAN_POINT ( 'NONE',  ( 35.16130328111002257, -282.0053857146162954, -279.4566598182844359 ) ) ;
#42794=CARTESIAN_POINT ( 'NONE',  ( -90.23014037448028546, -230.4905643893864351, -347.8797927120800750 ) ) ;
#42795=CARTESIAN_POINT ( 'NONE',  ( 201.9871895515903475, 295.7236489450776276, -54.00000000003252865 ) ) ;
#42796=CARTESIAN_POINT ( 'NONE',  ( -31.50900740967911418, -124.4314099722194271, -360.5826283136302095 ) ) ;
#42797=CARTESIAN_POINT ( 'NONE',  ( -103.3463686406470856, -272.1751947359218775, -238.8018806508005412 ) ) ;
#42798=CARTESIAN_POINT ( 'NONE',  ( -51.60821119650277211, -272.7858226493395932, -198.4015820285553104 ) ) ;
#42799=CARTESIAN_POINT ( 'NONE',  ( -30.60259167333858699, -294.4767486070976474, -347.0038692408732572 ) ) ;
#42800=CARTESIAN_POINT ( 'NONE',  ( 203.1405228849236551, 291.9636489450776367, -53.99999999998649258 ) ) ;
#42801=CARTESIAN_POINT ( 'NONE',  ( -38.33410824516327153, -272.7247879510630924, -193.8607035990392546 ) ) ;
#42802=CARTESIAN_POINT ( 'NONE',  ( -111.4467039188222230, -298.4695842586521621, -265.9663607470388342 ) ) ;
#42803=CARTESIAN_POINT ( 'NONE',  ( 22.37209593357130544, -289.4621960586882778, -313.2039241313341904 ) ) ;
#42804=CARTESIAN_POINT ( 'NONE',  ( -79.72055723569047814, -292.5441693620398951, -210.4803418033979483 ) ) ;
#42806=CARTESIAN_POINT ( 'NONE',  ( -99.81002242625292808, -296.8995688722610566, -315.0659762124039958 ) ) ;
#42807=CARTESIAN_POINT ( 'NONE',  ( 4.755710716422604456, -287.1299350248181668, -210.5849213593931779 ) ) ;
#42809=CARTESIAN_POINT ( 'NONE',  ( 36.94308322083536211, -294.6014360958367888, -290.0062136488913893 ) ) ;
#42810=CARTESIAN_POINT ( 'NONE',  ( -16.51750363910209529, -295.2825451050949823, -344.4830330095495015 ) ) ;
#42811=CARTESIAN_POINT ( 'NONE',  ( -6.043555356203813567, -292.6420092850357264, -204.3971571384788604 ) ) ;
#42813=CARTESIAN_POINT ( 'NONE',  ( -4.474996219834001643, -276.4019684744186520, -202.3094381367092183 ) ) ;
#42816=CARTESIAN_POINT ( 'NONE',  ( -113.2394910484469364, -277.9019554826218155, -282.9727093455488216 ) ) ;
#42817=CARTESIAN_POINT ( 'NONE',  ( -13.79106924338273465, -272.7628204906073961, -200.4196553217296355 ) ) ;
#42818=CARTESIAN_POINT ( 'NONE',  ( -40.80324115540862095, -275.0874032860800185, -197.0838641461715497 ) ) ;
#42819=CARTESIAN_POINT ( 'NONE',  ( 34.39746206246279314, -276.6870635009381090, -285.0886791179989928 ) ) ;
#42820=CARTESIAN_POINT ( 'NONE',  ( -52.36746971907324166, -275.6225641846683629, -195.8211480651992815 ) ) ;
#42821=CARTESIAN_POINT ( 'NONE',  ( 7.247075166880568631, -274.4684378754014915, -331.1731178007657945 ) ) ;
#42822=CARTESIAN_POINT ( 'NONE',  ( -110.4859856808060954, -297.1889233751873007, -271.4729337633568775 ) ) ;
#42823=CARTESIAN_POINT ( 'NONE',  ( 6.398713628329613989, -293.0198636074453589, -329.6035868868543730 ) ) ;
#42825=CARTESIAN_POINT ( 'NONE',  ( -91.01973036336205780, -279.8070895799918958, -215.1670064438016254 ) ) ;
#42826=CARTESIAN_POINT ( 'NONE',  ( 28.03144986521090942, -276.1606934816746843, -302.9612503922536462 ) ) ;
#42827=CARTESIAN_POINT ( 'NONE',  ( 36.22172509251311112, -285.9696824808132192, -249.1557035944968277 ) ) ;
#42828=CARTESIAN_POINT ( 'NONE',  ( -74.88680563515852384, -299.5540184192034872, -205.1830680766852595 ) ) ;
#42831=CARTESIAN_POINT ( 'NONE',  ( 34.67885154054003038, -286.9187211272819127, -283.2313108570337477 ) ) ;
#42832=CARTESIAN_POINT ( 'NONE',  ( -81.88003629483939960, -277.6761414321497341, -211.1840832710489053 ) ) ;
#42833=CARTESIAN_POINT ( 'NONE',  ( -68.75850763232951124, -278.2055545331609778, -203.8152005624672540 ) ) ;
#42834=CARTESIAN_POINT ( 'NONE',  ( 0.3791655890542534602, -284.5502087238114086, -335.2434396784627211 ) ) ;
#42835=CARTESIAN_POINT ( 'NONE',  ( -81.04357185737369207, -278.8659958423166927, -329.3295579403575175 ) ) ;
#42838=CARTESIAN_POINT ( 'NONE',  ( 32.98318290264681707, -273.5734388621735320, -240.8844823936609600 ) ) ;
#42840=CARTESIAN_POINT ( 'NONE',  ( 27.94861120575786373, -275.7579375589231745, -237.4815207562887736 ) ) ;
#42841=CARTESIAN_POINT ( 'NONE',  ( -1.233210700214557143, -284.5744958168110657, -336.3014604844067321 ) ) ;
#42842=DIRECTION ( 'NONE',  ( 1.000000000000000000, 0.000000000000000000, 0.000000000000000000 ) ) ;
#42843=CARTESIAN_POINT ( 'NONE',  ( -23.55030914826560107, -290.7974984251874844, -344.7049474779601610 ) ) ;
#42845=CARTESIAN_POINT ( 'NONE',  ( 32.09350561450776240, -291.1807039559618033, -241.8749988525930519 ) ) ;
#42846=CARTESIAN_POINT ( 'NONE',  ( 82.15178654341977449, -299.3244375900736713, -197.3535362759786835 ) ) ;
#42847=CARTESIAN_POINT ( 'NONE',  ( 30.63731071160582076, -273.8635672787256112, -242.2971858316740281 ) ) ;
#42848=CARTESIAN_POINT ( 'NONE',  ( 36.65378542668494788, -291.7690571875479009, -276.3221242687504287 ) ) ;
#42849=CARTESIAN_POINT ( 'NONE',  ( -32.04911714649202992, -124.5213432794980974, -365.6788127701597659 ) ) ;
#42851=CARTESIAN_POINT ( 'NONE',  ( -82.45843028957040133, -288.1358173262731270, -331.9012545646234571 ) ) ;
#42852=CARTESIAN_POINT ( 'NONE',  ( -110.2859365582050231, -286.0017888001420374, -281.8945940015221368 ) ) ;
#42853=CARTESIAN_POINT ( 'NONE',  ( 23.90004626481771766, -285.1865775561024066, -225.3786490164402210 ) ) ;
#42855=CARTESIAN_POINT ( 'NONE',  ( -71.66777297915450617, -284.9403834014049721, -335.4540948770547288 ) ) ;
#42856=CARTESIAN_POINT ( 'NONE',  ( -56.35102821920244764, -284.1062871213039784, -341.0098771506539492 ) ) ;
#42857=CARTESIAN_POINT ( 'NONE',  ( -109.6608862924576044, -292.8034163520489983, -249.1870272947481340 ) ) ;
#42858=CARTESIAN_POINT ( 'NONE',  ( -60.86869637794331567, -274.0883946869938086, -197.0100400529091473 ) ) ;
#42860=CARTESIAN_POINT ( 'NONE',  ( -96.18437910901727150, -287.9842961317706340, -317.7825145594953824 ) ) ;
#42861=CARTESIAN_POINT ( 'NONE',  ( 10.52605788214132154, -276.4120786065170705, -330.7423672093166829 ) ) ;
#42862=CARTESIAN_POINT ( 'NONE',  ( 24.30532809127641869, -296.1058158920566257, -312.5406284699500929 ) ) ;
#42864=FACE_OUTER_BOUND ( 'NONE', #80784, .T. ) ;
#42865=CARTESIAN_POINT ( 'NONE',  ( -108.2413029426609654, -282.9824654957402572, -289.7604109493443048 ) ) ;
#42866=CARTESIAN_POINT ( 'NONE',  ( -100.2006986490436731, -277.1047367086743520, -229.3557369658782363 ) ) ;
#42867=CARTESIAN_POINT ( 'NONE',  ( -73.59820918239149989, -272.0602176772786720, -203.1594538849116134 ) ) ;
#42868=CARTESIAN_POINT ( 'NONE',  ( 3.183731583561480782, -275.8402037402388487, -331.2017462877410026 ) ) ;
#42869=CARTESIAN_POINT ( 'NONE',  ( -34.85307546490108876, -293.6041043838564519, -196.7098145236149094 ) ) ;
#42871=CARTESIAN_POINT ( 'NONE',  ( 23.13404728551412859, -295.0673433039234510, -311.7546906606428365 ) ) ;
#42872=CARTESIAN_POINT ( 'NONE',  ( -93.31716609715077482, -297.1515798906043528, -322.5344633410979327 ) ) ;
#42873=CARTESIAN_POINT ( 'NONE',  ( -88.50336334515367298, -295.6271232538553022, -322.5040731885257514 ) ) ;
#42874=CARTESIAN_POINT ( 'NONE',  ( -2.412844464871696015, -290.5905754310778661, -336.7886395665131545 ) ) ;
#42875=CARTESIAN_POINT ( 'NONE',  ( -111.1073664436834036, -284.4412001287362841, -292.4891653028661835 ) ) ;
#42876=CARTESIAN_POINT ( 'NONE',  ( 17.21685270776070453, -272.9595542096821532, -217.7151634921682160 ) ) ;
#42877=CARTESIAN_POINT ( 'NONE',  ( 36.69181147680444610, -287.1179910019855015, -249.0048385730078451 ) ) ;
#42878=CARTESIAN_POINT ( 'NONE',  ( -43.31410954173887973, -279.1078519910307136, -344.7666092365767554 ) ) ;
#42880=CARTESIAN_POINT ( 'NONE',  ( -81.61131448491130413, -284.4912235280290815, -212.0206543908765582 ) ) ;
#42881=CARTESIAN_POINT ( 'NONE',  ( -6.473536761631635272, -286.6465964805590261, -338.7142974442743935 ) ) ;
#42882=CARTESIAN_POINT ( 'NONE',  ( -79.37448608631180491, -205.8233151019928755, -350.8497528714748341 ) ) ;
#42883=CARTESIAN_POINT ( 'NONE',  ( 35.69121543308865796, -287.1047188554355216, -273.7689465134058651 ) ) ;
#42884=CARTESIAN_POINT ( 'NONE',  ( -30.22473844818456357, -283.9054366481393572, -346.7952011474077381 ) ) ;
#42885=CARTESIAN_POINT ( 'NONE',  ( -110.5610600959339109, -289.3182681583547264, -293.5944727907153720 ) ) ;
#42886=CARTESIAN_POINT ( 'NONE',  ( -88.41054561962432956, -280.9504540514101336, -213.8066006221476414 ) ) ;
#42887=CARTESIAN_POINT ( 'NONE',  ( -111.9994805814217358, -279.6568818455803012, -287.0797929562136233 ) ) ;
#42888=CARTESIAN_POINT ( 'NONE',  ( -102.1549058820770313, -278.8436013845753223, -236.6617011701434308 ) ) ;
#42889=CARTESIAN_POINT ( 'NONE',  ( 3.816305524780818192, -276.5886482863444371, -208.0268477078438707 ) ) ;
#42890=CARTESIAN_POINT ( 'NONE',  ( -66.92443877691647458, -295.4292553076091963, -341.4658364154426522 ) ) ;
#42891=CARTESIAN_POINT ( 'NONE',  ( -48.32741492145277107, -287.2126116271723504, -344.2452685054324775 ) ) ;
#42892=CARTESIAN_POINT ( 'NONE',  ( -58.73382057611257778, -293.3800933243644522, -197.2255069819435107 ) ) ;
#42893=CARTESIAN_POINT ( 'NONE',  ( -86.70823585455920579, -294.6784618484621774, -324.5567933012786170 ) ) ;
#42895=CARTESIAN_POINT ( 'NONE',  ( -48.52128163487829227, -285.1157406284925173, -343.9568458006870060 ) ) ;
#42896=CARTESIAN_POINT ( 'NONE',  ( -82.37618502459633874, -295.3529007634854224, -327.9058686986957127 ) ) ;
#42898=CARTESIAN_POINT ( 'NONE',  ( -16.72298824514130544, -293.3921252007368139, -196.4939315650624962 ) ) ;
#42899=CARTESIAN_POINT ( 'NONE',  ( -5.521611183031291503, -281.1335980485591790, -204.5479383897285572 ) ) ;
#42900=CARTESIAN_POINT ( 'NONE',  ( 34.50576104723774762, -274.2678593768389419, -243.3284981473337609 ) ) ;
#42901=CARTESIAN_POINT ( 'NONE',  ( -99.78264212630969610, -290.6076096185357756, -315.2662054179045867 ) ) ;
#42902=CARTESIAN_POINT ( 'NONE',  ( -41.52501825401223812, -281.2437586226697022, -346.0618299537993607 ) ) ;
#42903=CARTESIAN_POINT ( 'NONE',  ( -111.2130690139982363, -291.1570712332410267, -248.7101330057250550 ) ) ;
#42904=CARTESIAN_POINT ( 'NONE',  ( 1.326375618783227850, -288.8532051437279620, -332.3035703458917851 ) ) ;
#42907=CARTESIAN_POINT ( 'NONE',  ( 187.6632728099119163, 270.6806713873519925, -138.5576046993855641 ) ) ;
#42908=CARTESIAN_POINT ( 'NONE',  ( 25.76221782734146259, -24.23989497703301410, -341.4211288899717260 ) ) ;
#42909=CARTESIAN_POINT ( 'NONE',  ( -110.4542110544635705, -276.2666405000204009, -253.6410175316879361 ) ) ;
#42910=CARTESIAN_POINT ( 'NONE',  ( -71.00689152637446000, -278.7932045549755458, -205.3911950726002829 ) ) ;
#42912=CARTESIAN_POINT ( 'NONE',  ( -89.68469539043113059, -278.2130118908750092, -218.9624251354857449 ) ) ;
#42913=CARTESIAN_POINT ( 'NONE',  ( -34.09983670283958190, -273.7586009658424473, -193.4505555537735404 ) ) ;
#42914=CARTESIAN_POINT ( 'NONE',  ( 202.9506381746226964, 290.1764997590596522, -82.60574211335169537 ) ) ;
#42915=CARTESIAN_POINT ( 'NONE',  ( -106.8753343450615603, -277.5364059179576088, -238.5528845538613325 ) ) ;
#42916=CARTESIAN_POINT ( 'NONE',  ( -64.68074490423430234, -281.4310051301540057, -339.8191875927582259 ) ) ;
#42918=CARTESIAN_POINT ( 'NONE',  ( -107.4315582720668658, -297.9324548610582610, -299.8465788017890645 ) ) ;
#42919=CARTESIAN_POINT ( 'NONE',  ( 21.85088651770049495, -293.4455971006245250, -227.5119796135670640 ) ) ;
#42921=CARTESIAN_POINT ( 'NONE',  ( 3.877436323619794845, -287.1694396218067595, -331.2683967500805124 ) ) ;
#42922=CARTESIAN_POINT ( 'NONE',  ( 39.45200817147964045, -276.1419123510364102, -265.4380250903752199 ) ) ;
#42923=CARTESIAN_POINT ( 'NONE',  ( -65.57467526137273239, -297.8390559024335289, -203.0417365263949421 ) ) ;
#42931=CARTESIAN_POINT ( 'NONE',  ( 33.75199499355257871, -282.3961663640185975, -252.4240552494830752 ) ) ;
#42932=CARTESIAN_POINT ( 'NONE',  ( -36.78281895853255179, -281.8192216275961641, -194.3636298791198556 ) ) ;
#42933=CARTESIAN_POINT ( 'NONE',  ( -71.52930925438678855, -282.5742416847735967, -335.1269718786251701 ) ) ;
#42934=CARTESIAN_POINT ( 'NONE',  ( -54.80597981071409208, -281.6858450058968515, -198.1563566814682815 ) ) ;
#42935=CARTESIAN_POINT ( 'NONE',  ( 27.25350221472448453, -273.5508280096681801, -234.7840550110153117 ) ) ;
#42938=CARTESIAN_POINT ( 'NONE',  ( -34.28725863740594093, -277.8174912846646407, -347.1389090946245801 ) ) ;
#42942=CARTESIAN_POINT ( 'NONE',  ( -25.87643237476757108, -275.4835837692420455, -345.9068255176592288 ) ) ;
#42945=CARTESIAN_POINT ( 'NONE',  ( -112.6832232484200489, -286.5723303095733741, -267.2089083834201801 ) ) ;
#42946=CARTESIAN_POINT ( 'NONE',  ( 33.60013994905521884, -292.9848324578926508, -288.2456658919263077 ) ) ;
#42947=ADVANCED_FACE ( 'NONE', ( #18504 ), #79449, .F. ) ;
#42948=CARTESIAN_POINT ( 'NONE',  ( -26.16757483272246532, -288.2620413764751675, -346.4429930266928750 ) ) ;
#42949=CARTESIAN_POINT ( 'NONE',  ( -39.98801080995787771, -284.2583033967503638, -196.3951051445042140 ) ) ;
#42950=CARTESIAN_POINT ( 'NONE',  ( -108.6687875047125829, -282.8898179301163509, -288.4669602723273556 ) ) ;
#42951=CARTESIAN_POINT ( 'NONE',  ( -37.28949761074304803, -287.2913482865603783, -344.3744363224035396 ) ) ;
#42952=CARTESIAN_POINT ( 'NONE',  ( 33.71175347916113907, -282.9994086819663721, -288.8106028473095535 ) ) ;
#42953=CARTESIAN_POINT ( 'NONE',  ( -46.60797950018415747, -271.9343522617085114, -195.9357411689216804 ) ) ;
#42954=CARTESIAN_POINT ( 'NONE',  ( -105.9498827348500498, -283.3819235057654282, -237.2045546385099897 ) ) ;
#42955=CARTESIAN_POINT ( 'NONE',  ( -91.24150544929607065, -297.8187481375996413, -322.5129313227120633 ) ) ;
#42956=CARTESIAN_POINT ( 'NONE',  ( -68.99698313679613193, -283.6367567159081204, -202.1710632356213750 ) ) ;
#42957=CARTESIAN_POINT ( 'NONE',  ( -104.6630564907187306, -279.8794624052123936, -241.5298255218714587 ) ) ;
#42958=CARTESIAN_POINT ( 'NONE',  ( 32.35228777691182955, -289.9200825889580528, -298.6561603426944771 ) ) ;
#42961=CARTESIAN_POINT ( 'NONE',  ( 26.89486623655271913, -296.0036506589205487, -310.2461187141660730 ) ) ;
#42963=CARTESIAN_POINT ( 'NONE',  ( -96.87572181362651236, -275.9274016452608862, -315.9758186221450842 ) ) ;
#42964=CARTESIAN_POINT ( 'NONE',  ( -110.6309313194398811, -289.4566652400316684, -293.6185062433973485 ) ) ;
#42965=CARTESIAN_POINT ( 'NONE',  ( -76.09530833945771633, -293.9787772851444174, -333.2267423522411605 ) ) ;
#42966=CARTESIAN_POINT ( 'NONE',  ( -22.07572759736078538, -278.9365094385113366, -198.4187589170627746 ) ) ;
#42967=CARTESIAN_POINT ( 'NONE',  ( -109.3263870912830953, -270.8798442382307030, -251.2027108781749689 ) ) ;
#42968=CARTESIAN_POINT ( 'NONE',  ( -107.4772215038594823, -292.1569183094522373, -248.3584528825911093 ) ) ;
#42969=CARTESIAN_POINT ( 'NONE',  ( 39.58706461736020543, -284.0519495502702512, -270.3284710469133074 ) ) ;
#42970=CARTESIAN_POINT ( 'NONE',  ( -66.67596205403893350, -293.9093788545202983, -340.8181409362580894 ) ) ;
#42971=CARTESIAN_POINT ( 'NONE',  ( -53.56477480331713537, -290.8639117648802994, -342.3559251638833416 ) ) ;
#42972=CARTESIAN_POINT ( 'NONE',  ( -64.01186305909970997, -289.9490158890015437, -199.1532044938730621 ) ) ;
#42973=CARTESIAN_POINT ( 'NONE',  ( -5.521347270807003049, -290.0503953247497293, -336.7150181181185076 ) ) ;
#42975=CARTESIAN_POINT ( 'NONE',  ( -100.4380457336314834, -290.8464015569286971, -307.4940090770277266 ) ) ;
#42977=CARTESIAN_POINT ( 'NONE',  ( -112.7397341039777956, -291.5861654050265770, -283.9682415960828052 ) ) ;
#42978=CARTESIAN_POINT ( 'NONE',  ( 5.275257023345053753, -278.6457423904747088, -208.2145029204482967 ) ) ;
#42979=CARTESIAN_POINT ( 'NONE',  ( -106.9520964504961853, -290.2587069915728080, -292.5145035144574308 ) ) ;
#42981=CARTESIAN_POINT ( 'NONE',  ( -39.59089506606640185, -280.3579449401496504, -193.4020806963975758 ) ) ;
#42982=CARTESIAN_POINT ( 'NONE',  ( 23.38362003892255103, -281.8513012658209504, -317.6918225101389339 ) ) ;
#42983=CARTESIAN_POINT ( 'NONE',  ( 36.73057395195334607, -285.7040377109205451, -282.2028423213719179 ) ) ;
#42985=CARTESIAN_POINT ( 'NONE',  ( 27.93003924501046242, -280.1662176731669547, -305.7230398334868369 ) ) ;
#42986=CARTESIAN_POINT ( 'NONE',  ( -112.1547656182552544, -282.6287637653284719, -264.3816528938895090 ) ) ;
#42987=DIRECTION ( 'NONE',  ( -1.000000000000000000, -0.000000000000000000, -0.000000000000000000 ) ) ;
#42988=CARTESIAN_POINT ( 'NONE',  ( -109.0915178644586518, -276.6992410593323939, -296.4902368657858460 ) ) ;
#42990=CARTESIAN_POINT ( 'NONE',  ( -113.1796386647707209, -283.6201004365038898, -258.6052285045099666 ) ) ;
#42991=CARTESIAN_POINT ( 'NONE',  ( -56.91462729414405430, -274.5961634143266110, -199.8135862455631866 ) ) ;
#42993=CARTESIAN_POINT ( 'NONE',  ( -28.02533708165118043, -293.7723706814070397, -197.1002125915819363 ) ) ;
#42994=CARTESIAN_POINT ( 'NONE',  ( 37.60797985208085947, -277.1648375924737024, -285.2322902752480331 ) ) ;
#42995=CARTESIAN_POINT ( 'NONE',  ( -8.734304219170786254, -276.3339693611055736, -337.5587720912180316 ) ) ;
#42996=CARTESIAN_POINT ( 'NONE',  ( 13.73507041340559987, -296.3369496267696377, -325.3519369297682715 ) ) ;
#42997=CARTESIAN_POINT ( 'NONE',  ( -87.38282391052821652, -289.8941038545590914, -328.9536744273229942 ) ) ;
#42998=AXIS2_PLACEMENT_3D ( 'NONE', #93164, #14113, #79888 ) ;
#42999=CARTESIAN_POINT ( 'NONE',  ( 38.20202039902547142, -279.5909893032552986, -267.1435502085005282 ) ) ;
#43001=CARTESIAN_POINT ( 'NONE',  ( 22.21060817566707613, -292.7300162469010161, -221.5500272323206730 ) ) ;
#43002=CARTESIAN_POINT ( 'NONE',  ( -104.9155595301911177, -289.9899980931524510, -241.9947906946783860 ) ) ;
#43003=CARTESIAN_POINT ( 'NONE',  ( -76.07183415066907628, -293.5689970976574728, -334.6475355771692648 ) ) ;
#43006=CARTESIAN_POINT ( 'NONE',  ( -70.24281893392146969, -291.1139922498899750, -205.1268875266394502 ) ) ;
#43008=CARTESIAN_POINT ( 'NONE',  ( 30.91033621190086578, -272.8380690714490129, -254.8156830097664738 ) ) ;
#43009=CARTESIAN_POINT ( 'NONE',  ( -113.9996203384661442, -295.5487917682976331, -275.3122152630396613 ) ) ;
#43010=CARTESIAN_POINT ( 'NONE',  ( -112.0399466478455395, -285.6591695094882652, -286.8980536679063675 ) ) ;
#43011=CARTESIAN_POINT ( 'NONE',  ( 18.66312710380852735, -286.7206643520017906, -223.5179380335132464 ) ) ;
#43012=CARTESIAN_POINT ( 'NONE',  ( 33.18551471823606391, -277.3530738039769403, -291.7735628420287526 ) ) ;
#43013=CARTESIAN_POINT ( 'NONE',  ( 13.45615586511399364, -292.3575378159243883, -325.1258565047109528 ) ) ;
#43014=CARTESIAN_POINT ( 'NONE',  ( 36.43631108011300057, -295.3890312197223693, -276.2584965499544865 ) ) ;
#43016=CARTESIAN_POINT ( 'NONE',  ( 35.98454281686093026, -274.2915732756347325, -266.1313019239624964 ) ) ;
#43019=CARTESIAN_POINT ( 'NONE',  ( -110.3270113682650191, -295.9106256597181641, -294.8333192457906762 ) ) ;
#43020=CARTESIAN_POINT ( 'NONE',  ( -20.78575138063733618, -290.7581399825188555, -342.9366975940424140 ) ) ;
#43021=CARTESIAN_POINT ( 'NONE',  ( 201.0378816431136215, 294.4824024966172828, -54.00000000000627409 ) ) ;
#43022=CARTESIAN_POINT ( 'NONE',  ( -36.91288064764863464, -299.1370683167476159, -193.6701508778304799 ) ) ;
#43023=CARTESIAN_POINT ( 'NONE',  ( -0.9334829628409744284, -289.2068616029832242, -333.8097212761984451 ) ) ;
#43025=CARTESIAN_POINT ( 'NONE',  ( -84.41316979716314961, -278.4811890448138456, -209.6547865246078572 ) ) ;
#43026=CARTESIAN_POINT ( 'NONE',  ( 26.43185067494878382, -294.7704193162263095, -313.3290944831168190 ) ) ;
#43027=CARTESIAN_POINT ( 'NONE',  ( -77.50208864386091534, -287.7240688354767144, -334.6675509583748749 ) ) ;
#43028=CARTESIAN_POINT ( 'NONE',  ( -53.28072217516110243, -295.5843197245558258, -345.7262813025665764 ) ) ;
#43029=CARTESIAN_POINT ( 'NONE',  ( 19.35952538546157342, -293.2344275275639234, -224.3298394215769918 ) ) ;
#43033=CARTESIAN_POINT ( 'NONE',  ( 39.00903594524251616, -289.0869142496551945, -271.5212520357966923 ) ) ;
#43034=CARTESIAN_POINT ( 'NONE',  ( -19.11405058567864046, -286.3380690714489560, -350.3683826091709648 ) ) ;
#43036=CARTESIAN_POINT ( 'NONE',  ( -19.77144108156758762, -279.6207711645471363, -195.4425501615428118 ) ) ;
#43037=CARTESIAN_POINT ( 'NONE',  ( -1.529447730817133699, -284.5764642505654933, -336.0835382243644744 ) ) ;
#43038=CARTESIAN_POINT ( 'NONE',  ( -113.6214010409390198, -283.0601168966554724, -275.6587063939135760 ) ) ;
#43039=CARTESIAN_POINT ( 'NONE',  ( 15.08045641260617131, -286.3852148179146297, -323.2121510886523197 ) ) ;
#43040=CARTESIAN_POINT ( 'NONE',  ( 7.528913281278284408, -278.3081279420530905, -331.4747033965260812 ) ) ;
#43041=CARTESIAN_POINT ( 'NONE',  ( -65.82530665041743134, -274.0022405054091905, -203.1244341982884407 ) ) ;
#43043=CARTESIAN_POINT ( 'NONE',  ( -99.46773070686191431, -279.0818708372468109, -231.9325004426448800 ) ) ;
#43044=CARTESIAN_POINT ( 'NONE',  ( -110.4528495135877080, -277.9332010092538781, -267.8965625832013302 ) ) ;
#43045=CARTESIAN_POINT ( 'NONE',  ( 17.85751899607230087, -275.8991674616297018, -217.0445142784453765 ) ) ;
#43046=CARTESIAN_POINT ( 'NONE',  ( -113.9802245218702268, -277.3676166370366332, -268.7273205219454439 ) ) ;
#43047=CARTESIAN_POINT ( 'NONE',  ( -95.96838508513684474, -238.3309465572374393, -339.6183069132351875 ) ) ;
#43048=CARTESIAN_POINT ( 'NONE',  ( -81.51615232335547034, -297.0651251487017817, -332.7733388738899976 ) ) ;
#43049=CARTESIAN_POINT ( 'NONE',  ( -37.37352853689063892, -288.5519495502701943, -195.3611179825600175 ) ) ;
#43050=ORIENTED_EDGE ( 'NONE', *, *, #40194, .F. ) ;
#43052=CARTESIAN_POINT ( 'NONE',  ( -39.99883305194413197, -287.0976569310942068, -197.1001753257822031 ) ) ;
#43053=CARTESIAN_POINT ( 'NONE',  ( -75.61595190626032092, -287.3093675063864794, -204.6571186150938502 ) ) ;
#43054=CARTESIAN_POINT ( 'NONE',  ( -3.326323417341269906, -287.9394320132768712, -335.1230247582908532 ) ) ;
#43055=CARTESIAN_POINT ( 'NONE',  ( -114.0899685434597757, -284.1363342471523765, -264.2468811833574023 ) ) ;
#43056=CARTESIAN_POINT ( 'NONE',  ( 0.8310072182383487771, -278.9699686352900585, -207.1411680245042817 ) ) ;
#43057=CARTESIAN_POINT ( 'NONE',  ( -37.30363014210946915, -287.9130126734615374, -196.1132745426634472 ) ) ;
#43058=CARTESIAN_POINT ( 'NONE',  ( 5.340325040149338065, -279.1214896391054481, -210.2865603197639075 ) ) ;
#43059=CARTESIAN_POINT ( 'NONE',  ( -54.04987631655905744, -278.5862322817555992, -341.9823189662692471 ) ) ;
#43060=CARTESIAN_POINT ( 'NONE',  ( 26.82379824955405567, -276.5222960395601035, -305.4065193446833746 ) ) ;
#43061=CARTESIAN_POINT ( 'NONE',  ( -1.997644142801269229, -287.3895289439580552, -338.3229192107883705 ) ) ;
#43062=CARTESIAN_POINT ( 'NONE',  ( -94.27262595806554657, -284.6522828767522810, -321.9851690422206048 ) ) ;
#43063=CARTESIAN_POINT ( 'NONE',  ( -1.657110631631045328, -283.0843707216288294, -338.5236955151176517 ) ) ;
#43066=FACE_BOUND ( 'NONE', #6007, .T. ) ;
#43067=CARTESIAN_POINT ( 'NONE',  ( -88.63751928321207174, -291.6232937575563824, -326.1199237050473698 ) ) ;
#43068=CARTESIAN_POINT ( 'NONE',  ( -109.9574927611636639, -289.5440281105414897, -246.1071680132189385 ) ) ;
#43070=CARTESIAN_POINT ( 'NONE',  ( -108.7617064387818147, -271.8239779507147773, -254.1564536063076787 ) ) ;
#43071=CARTESIAN_POINT ( 'NONE',  ( 36.26969031211439898, -293.1823233105158124, -292.7827458807917083 ) ) ;
#43072=CARTESIAN_POINT ( 'NONE',  ( -23.67540736367092435, -287.3543498106038214, -342.8283602820863507 ) ) ;
#43073=CARTESIAN_POINT ( 'NONE',  ( 36.63486155438262415, -291.7616501970875902, -268.0282372174906413 ) ) ;
#43074=CARTESIAN_POINT ( 'NONE',  ( -8.045972640272154308, -289.8648491861502521, -337.7124921573010283 ) ) ;
#43075=CARTESIAN_POINT ( 'NONE',  ( -110.4542110544635705, -298.8376638359844719, -287.0812184334320705 ) ) ;
#43076=CARTESIAN_POINT ( 'NONE',  ( 35.87812805681895867, -289.7616302273697215, -286.6635252069625039 ) ) ;
#43077=CARTESIAN_POINT ( 'NONE',  ( -72.55183474986085912, -289.5870430541191354, -203.9366749534805479 ) ) ;
#43078=CARTESIAN_POINT ( 'NONE',  ( -101.7150847837339143, -293.0686206528743014, -231.7766073015210111 ) ) ;
#43079=CARTESIAN_POINT ( 'NONE',  ( -108.5972248506468389, -285.7164599226876476, -253.3938026246506183 ) ) ;
#43080=CARTESIAN_POINT ( 'NONE',  ( 35.63574586544919498, -295.3215238158265947, -252.3522088893608952 ) ) ;
#43081=CARTESIAN_POINT ( 'NONE',  ( -112.3417001281054723, -270.5523139186827279, -270.3356821209761165 ) ) ;
#43083=CARTESIAN_POINT ( 'NONE',  ( -89.05288204568653043, -275.3098263147451235, -215.4777901952105026 ) ) ;
#43085=CARTESIAN_POINT ( 'NONE',  ( -8.439839163762631102, -281.8610033199269651, -337.5718623625680266 ) ) ;
#43086=CARTESIAN_POINT ( 'NONE',  ( -51.41756448579535999, -281.2318447457062121, -344.0814075003600010 ) ) ;
#43087=CARTESIAN_POINT ( 'NONE',  ( -56.04090144877764601, -294.4842382318693694, -344.8896272254696100 ) ) ;
#43088=CARTESIAN_POINT ( 'NONE',  ( 12.24178478955131588, -272.9929214192598579, -215.3425482218490572 ) ) ;
#43089=CARTESIAN_POINT ( 'NONE',  ( -101.8425540965401268, -276.1311249352486925, -307.6258920054404484 ) ) ;
#43090=CARTESIAN_POINT ( 'NONE',  ( -104.1739781119986645, -298.2783209675659464, -239.6658634530940617 ) ) ;
#43091=CARTESIAN_POINT ( 'NONE',  ( 34.64775987874817531, -295.1779223414953321, -285.6824479857635311 ) ) ;
#43093=CARTESIAN_POINT ( 'NONE',  ( -39.68398696466171316, -295.8851181770038465, -343.4975490098863702 ) ) ;
#43095=CARTESIAN_POINT ( 'NONE',  ( -5.446708689715258345, -284.4897839715625310, -202.0887492806195382 ) ) ;
#43096=CARTESIAN_POINT ( 'NONE',  ( -84.07483455525556337, -297.3891023827070512, -214.2146934236563709 ) ) ;
#43097=CARTESIAN_POINT ( 'NONE',  ( -94.39915396130795955, -283.8495799133680180, -322.0860597705161581 ) ) ;
#43098=CARTESIAN_POINT ( 'NONE',  ( 32.84385895012785284, -287.6228605759146149, -301.9796503380684953 ) ) ;
#43099=CARTESIAN_POINT ( 'NONE',  ( 22.73330092127427449, -296.1512816504139209, -315.8517879605568623 ) ) ;
#43100=CARTESIAN_POINT ( 'NONE',  ( 36.52767371428124932, -291.3968879094392150, -258.3081852475582423 ) ) ;
#43101=CARTESIAN_POINT ( 'NONE',  ( -77.39959017020464671, -278.7268106503487957, -204.7287682977936072 ) ) ;
#43102=CARTESIAN_POINT ( 'NONE',  ( -95.95921662488163406, -294.6952119285919025, -223.5744983911110353 ) ) ;
#43104=CARTESIAN_POINT ( 'NONE',  ( 32.22179632868873256, -286.0377678056952959, -246.9506402988595823 ) ) ;
#43107=CARTESIAN_POINT ( 'NONE',  ( -108.6135127068038315, -298.4030657779300668, -251.1611522022819543 ) ) ;
#43108=CARTESIAN_POINT ( 'NONE',  ( -22.69702909277681258, -281.6611815316325647, -195.3130139600934001 ) ) ;
#43109=CARTESIAN_POINT ( 'NONE',  ( -80.94103828022655023, -293.6605088080333417, -331.8862703230191755 ) ) ;
#43110=CARTESIAN_POINT ( 'NONE',  ( 30.33452865869570303, -281.9186277349919578, -297.7276679514509965 ) ) ;
#43111=CARTESIAN_POINT ( 'NONE',  ( -105.2546098419397396, -297.1890518288208796, -233.9597594180537214 ) ) ;
#43112=CARTESIAN_POINT ( 'NONE',  ( -80.14634731296082748, -298.9808505886986154, -210.3738699193686728 ) ) ;
#43113=CARTESIAN_POINT ( 'NONE',  ( 31.41209627129236992, -285.2222962678480940, -238.8945313818403520 ) ) ;
#43114=CARTESIAN_POINT ( 'NONE',  ( -109.8054437565513837, -280.8014833013458542, -250.9722235702734849 ) ) ;
#43115=CARTESIAN_POINT ( 'NONE',  ( -102.7370592014746080, -296.0582745058885052, -237.2807484572368253 ) ) ;
#43118=CARTESIAN_POINT ( 'NONE',  ( -64.63379755445335206, -285.3901504232107413, -339.8376479859867345 ) ) ;
#43120=CARTESIAN_POINT ( 'NONE',  ( -20.19161114001082069, -283.7666405000204009, -195.3683826091709363 ) ) ;
#43121=CARTESIAN_POINT ( 'NONE',  ( 33.56848811359044760, -274.3706063330832876, -240.6279754453531154 ) ) ;
#43124=CARTESIAN_POINT ( 'NONE',  ( 23.34242617102849238, -292.8219737722124023, -229.7848093798835976 ) ) ;
#43125=CARTESIAN_POINT ( 'NONE',  ( 34.12324776698246609, -282.8365456831581923, -252.3246610363836737 ) ) ;
#43126=CARTESIAN_POINT ( 'NONE',  ( 32.02057755700564456, -277.4862305546627681, -295.7151879516842996 ) ) ;
#43127=CARTESIAN_POINT ( 'NONE',  ( 31.67653161100110637, -283.5715295707567520, -302.7798371038574601 ) ) ;
#43128=CARTESIAN_POINT ( 'NONE',  ( 13.62179459227293776, -279.5800448321840577, -217.4712203547014155 ) ) ;
#43129=CARTESIAN_POINT ( 'NONE',  ( -86.82225947929823917, -281.3639507526208945, -213.9991193285531779 ) ) ;
#43130=CARTESIAN_POINT ( 'NONE',  ( 99.18597135844251511, -299.7172817242040992, -193.3609922739482556 ) ) ;
#43131=CARTESIAN_POINT ( 'NONE',  ( 33.71436872516444794, -275.0066564734262329, -240.5580124021094832 ) ) ;
#43132=CARTESIAN_POINT ( 'NONE',  ( 36.32943497150740342, -295.3342596619310143, -259.6897520325212554 ) ) ;
#43134=LINE ( 'NONE', #6699, #88922 ) ;
#43135=CARTESIAN_POINT ( 'NONE',  ( 28.48949586576387105, -292.1879562902235534, -307.9711640323280335 ) ) ;
#43136=CARTESIAN_POINT ( 'NONE',  ( -21.91492666388166199, -273.7628683894821506, -198.9468119792075811 ) ) ;
#43138=CARTESIAN_POINT ( 'NONE',  ( 20.76974850472888789, -294.3992066522878872, -220.8864631929152722 ) ) ;
#43139=CARTESIAN_POINT ( 'NONE',  ( -112.3452863284742875, -275.1604526064900824, -261.9424758988611188 ) ) ;
#43140=CARTESIAN_POINT ( 'NONE',  ( -40.63081006024501107, -293.2167509284273024, -193.8157199773786772 ) ) ;
#43141=CARTESIAN_POINT ( 'NONE',  ( -42.77214904491643210, -291.1208601627756138, -345.0490337553362679 ) ) ;
#43142=CARTESIAN_POINT ( 'NONE',  ( -90.40330567983866672, -275.8047274803942628, -323.2030369195602475 ) ) ;
#43143=CARTESIAN_POINT ( 'NONE',  ( -43.29841267956833661, -279.0481235032263498, -344.5624102469091099 ) ) ;
#43144=CARTESIAN_POINT ( 'NONE',  ( 2.316716786032549713, -292.5966299899486671, -333.4183780738695759 ) ) ;
#43145=CARTESIAN_POINT ( 'NONE',  ( 34.98932837053446576, -283.1246450727509227, -247.8105570810429299 ) ) ;
#43147=CARTESIAN_POINT ( 'NONE',  ( -109.7241501330076119, -283.6261508395967894, -258.6624437431430010 ) ) ;
#43149=CARTESIAN_POINT ( 'NONE',  ( 3.398499492847016690, -282.1547360494830059, -331.0219785869745124 ) ) ;
#43150=CARTESIAN_POINT ( 'NONE',  ( -39.59202080859100192, -281.1042144791311443, -193.6902528982587626 ) ) ;
#43151=CARTESIAN_POINT ( 'NONE',  ( -111.3336391416264775, -283.5989161604972537, -250.3325926131205108 ) ) ;
#43152=CARTESIAN_POINT ( 'NONE',  ( -94.79367732475492403, -280.1852755811136149, -219.4485406614516876 ) ) ;
#43153=SHAPE_REPRESENTATION_RELATIONSHIP ( 'NONE' , 'NONE' ,  #49383, #12545 ) ;
#43154=CARTESIAN_POINT ( 'NONE',  ( -98.23830774821144018, -279.4540776291964335, -316.3641934583372404 ) ) ;
#43155=CARTESIAN_POINT ( 'NONE',  ( -37.37352853689063181, -274.5523547857346784, -340.3611179825599606 ) ) ;
#43158=CARTESIAN_POINT ( 'NONE',  ( -40.63048489267862351, -300.0109735804684306, -195.4203633066897794 ) ) ;
#43159=CARTESIAN_POINT ( 'NONE',  ( -110.0949494014835466, -276.3561144569253543, -287.1154956881167095 ) ) ;
#43160=CARTESIAN_POINT ( 'NONE',  ( -111.3357030163400054, -292.5313809838983730, -253.0735052437564434 ) ) ;
#43161=CARTESIAN_POINT ( 'NONE',  ( 35.52537832964075193, -292.9778651859134015, -276.2161623890235660 ) ) ;
#43162=CARTESIAN_POINT ( 'NONE',  ( -112.5784700627718991, -290.2619637076062986, -254.2068949525582582 ) ) ;
#43164=CARTESIAN_POINT ( 'NONE',  ( 37.20503191951331701, -292.3390388943843163, -287.1948284796106918 ) ) ;
#43165=CARTESIAN_POINT ( 'NONE',  ( -75.11223442820546836, -283.9396528411556346, -206.9590111263654251 ) ) ;
#43166=CARTESIAN_POINT ( 'NONE',  ( -91.67919673014479542, -293.1278624160604522, -219.7626570154602632 ) ) ;
#43167=CARTESIAN_POINT ( 'NONE',  ( 9.485835014756968775, -285.1896870155832175, -213.4586601889024848 ) ) ;
#43168=CARTESIAN_POINT ( 'NONE',  ( -21.26412956754484895, -284.1569110213982299, -342.1264904004002574 ) ) ;
#43169=CARTESIAN_POINT ( 'NONE',  ( -43.15249233114293048, -290.0650829187710542, -346.9055815769275455 ) ) ;
#43170=CARTESIAN_POINT ( 'NONE',  ( 22.15997060491829629, -281.4527292910796632, -227.9637168623945058 ) ) ;
#43171=CARTESIAN_POINT ( 'NONE',  ( 38.84046996665242801, -292.4539969654507559, -278.8661077269548514 ) ) ;
#43172=CARTESIAN_POINT ( 'NONE',  ( -36.07922049771882200, -289.8395626299993069, -347.2023528754664312 ) ) ;
#43173=CARTESIAN_POINT ( 'NONE',  ( -112.8064066322788079, -290.8560805461020777, -285.4146964588423430 ) ) ;
#43174=CARTESIAN_POINT ( 'NONE',  ( -108.0291923993588341, -284.9594647674005046, -252.1326117100746274 ) ) ;
#43177=CARTESIAN_POINT ( 'NONE',  ( -25.08392384678993636, -296.7580026720443698, -345.1809718579603441 ) ) ;
#43178=CARTESIAN_POINT ( 'NONE',  ( -74.38238042461829025, -294.2185329525826774, -337.3628643076092430 ) ) ;
#43179=CARTESIAN_POINT ( 'NONE',  ( -94.96859516353185882, -278.2462975274661403, -225.1463653065975734 ) ) ;
#43180=CARTESIAN_POINT ( 'NONE',  ( -70.09986567011543457, -273.1397759288119573, -200.7304146571214005 ) ) ;
#43181=CARTESIAN_POINT ( 'NONE',  ( -41.09370002469045602, -293.5800674306174187, -343.9715643559873115 ) ) ;
#43182=CARTESIAN_POINT ( 'NONE',  ( 35.16168541606742082, -277.5058202653120247, -285.2350246849453015 ) ) ;
#43183=CARTESIAN_POINT ( 'NONE',  ( -103.1140283917687839, -271.1537135675578156, -235.8279615827835869 ) ) ;
#43184=CARTESIAN_POINT ( 'NONE',  ( 15.14880353323818518, -294.0182675175411759, -218.9865118218939699 ) ) ;
#43185=CARTESIAN_POINT ( 'NONE',  ( -93.30952029014373750, -296.9615348438026103, -317.7285187922821024 ) ) ;
#43187=CARTESIAN_POINT ( 'NONE',  ( -100.7557193666334996, -295.0938930831584344, -230.0040790715417245 ) ) ;
#43188=CARTESIAN_POINT ( 'NONE',  ( -36.90591992003509603, -298.7088833530352758, -193.4630033034831627 ) ) ;
#43189=CARTESIAN_POINT ( 'NONE',  ( 34.58274047468821522, -286.3312780081349729, -285.9845234415230948 ) ) ;
#43190=CARTESIAN_POINT ( 'NONE',  ( -36.74506159037600383, -276.0598066130880284, -195.3507321840570228 ) ) ;
#43191=CARTESIAN_POINT ( 'NONE',  ( -78.29610070260136467, -290.5590415597208676, -331.1357981330311873 ) ) ;
#43192=CARTESIAN_POINT ( 'NONE',  ( -106.7903684750227740, -273.4693186665585358, -237.2490451406089562 ) ) ;
#43193=CARTESIAN_POINT ( 'NONE',  ( -75.66554140224893388, -295.9118751780163166, -332.5760849177794967 ) ) ;
#43194=CARTESIAN_POINT ( 'NONE',  ( -99.10266487916675260, -279.9488245874191534, -313.5350688882363102 ) ) ;
#43195=CARTESIAN_POINT ( 'NONE',  ( -113.8840718870465025, -277.2575360720655908, -268.7279513365879779 ) ) ;
#43196=CARTESIAN_POINT ( 'NONE',  ( -71.70064926505257574, -282.8428543491347682, -339.1562878804249976 ) ) ;
#43197=CARTESIAN_POINT ( 'NONE',  ( 23.55720624841553956, -274.2730564956050330, -223.3861306643977969 ) ) ;
#43198=CARTESIAN_POINT ( 'NONE',  ( -35.33644442437506683, -278.4767734867814397, -194.1745045521862210 ) ) ;
#43199=CARTESIAN_POINT ( 'NONE',  ( 21.45751705949315991, -278.9096077347263076, -223.5145792692347300 ) ) ;
#43200=CARTESIAN_POINT ( 'NONE',  ( -93.98298991252788426, -295.8966078572881884, -223.5119845526984079 ) ) ;
#43201=CARTESIAN_POINT ( 'NONE',  ( 4.028684547046823106, -278.4954588719372168, -332.9805170302796000 ) ) ;
#43203=CARTESIAN_POINT ( 'NONE',  ( 7.884347619584023192, -290.6862075724064880, -210.0215106034997632 ) ) ;
#43204=CARTESIAN_POINT ( 'NONE',  ( -3.321352055266363124, -292.4889651421707981, -201.2696962055109395 ) ) ;
#43205=CARTESIAN_POINT ( 'NONE',  ( 14.73801679728006953, -276.7838768352112311, -216.1602738029803277 ) ) ;
#43206=CARTESIAN_POINT ( 'NONE',  ( -47.49694680946925018, -295.9227495756036888, -196.1675456646217128 ) ) ;
#43207=CARTESIAN_POINT ( 'NONE',  ( -89.76858360487166522, -284.5322756325821842, -214.1142050115937252 ) ) ;
#43208=( NAMED_UNIT ( * ) SI_UNIT ( $, .STERADIAN. ) SOLID_ANGLE_UNIT ( ) );
#43209=CARTESIAN_POINT ( 'NONE',  ( -101.3525388959677542, -282.0267410142292306, -309.5440909481995959 ) ) ;
#43212=CARTESIAN_POINT ( 'NONE',  ( -9.563045460428373445, -291.2181804358820614, -202.3697337995337193 ) ) ;
#43213=CARTESIAN_POINT ( 'NONE',  ( -37.25605685649913568, -284.1927833791692137, -196.1133150158942442 ) ) ;
#43216=CARTESIAN_POINT ( 'NONE',  ( 22.09296495084021217, -292.1788802303631769, -316.1262207855465931 ) ) ;
#43217=CARTESIAN_POINT ( 'NONE',  ( -108.6619060583244618, -282.6838120222776638, -297.6402818262262713 ) ) ;
#43218=CARTESIAN_POINT ( 'NONE',  ( -26.88827593870426114, -278.5171435650348712, -343.4170303822178880 ) ) ;
#43219=CARTESIAN_POINT ( 'NONE',  ( -111.1049538694434062, -285.4969461246036531, -291.0248813545133544 ) ) ;
#43220=CARTESIAN_POINT ( 'NONE',  ( -5.798649145682235329, -286.4787492498483630, -204.5139387041926113 ) ) ;
#43221=CARTESIAN_POINT ( 'NONE',  ( -94.90266296159016690, -279.3348759963886891, -316.2300187250377803 ) ) ;
#43222=CARTESIAN_POINT ( 'NONE',  ( -89.59605644901319010, -280.0952124059233483, -219.0830218228622925 ) ) ;
#43224=CARTESIAN_POINT ( 'NONE',  ( -60.03904446582659205, -287.7394642787486418, -198.4510519825464883 ) ) ;
#43226=CARTESIAN_POINT ( 'NONE',  ( 19.39083834128441808, -298.5773980873777305, -193.3626504022654160 ) ) ;
#43227=CARTESIAN_POINT ( 'NONE',  ( -69.44299170516677577, -291.4566251049550942, -337.7506860642808988 ) ) ;
#43229=CARTESIAN_POINT ( 'NONE',  ( -19.11405058567862625, -288.7662352645559167, -190.3538533559490702 ) ) ;
#43231=CARTESIAN_POINT ( 'NONE',  ( 3.879575505991686324, -272.6051628109363492, -207.4436833820658705 ) ) ;
#43233=CARTESIAN_POINT ( 'NONE',  ( 25.83694142330487864, -292.5192410161683370, -312.9627572360799945 ) ) ;
#43234=CARTESIAN_POINT ( 'NONE',  ( 32.92894111148237357, -288.7802857845354083, -248.1210532869659460 ) ) ;
#43235=CARTESIAN_POINT ( 'NONE',  ( -8.878075120584858482, -282.1898331116839245, -202.0398470186532052 ) ) ;
#43236=CARTESIAN_POINT ( 'NONE',  ( 24.21771394611131711, -288.3714762427218830, -225.0947415768949043 ) ) ;
#43237=CARTESIAN_POINT ( 'NONE',  ( 37.34719363658153668, -289.0767546778642441, -287.0001107046767288 ) ) ;
#43238=CARTESIAN_POINT ( 'NONE',  ( -72.31965602083955957, -285.5151786706056782, -336.7052454764717595 ) ) ;
#43239=CARTESIAN_POINT ( 'NONE',  ( -107.4200032711850668, -279.1281020763574929, -238.3261315319869311 ) ) ;
#43241=CARTESIAN_POINT ( 'NONE',  ( -25.16444040404978466, -292.9780412936349308, -344.9864740904712903 ) ) ;
#43242=CARTESIAN_POINT ( 'NONE',  ( 26.72070855840134840, -281.9477855309365850, -313.0812279752951781 ) ) ;
#43243=CARTESIAN_POINT ( 'NONE',  ( 53.85457608967112719, -301.1225409177318966, -195.8910045484337559 ) ) ;
#43244=CARTESIAN_POINT ( 'NONE',  ( 10.59707575819634329, -295.1948066931273615, -210.1954327657594490 ) ) ;
#43245=CARTESIAN_POINT ( 'NONE',  ( -24.31103652693491313, -272.4560338893585367, -195.4466184879564423 ) ) ;
#43247=CARTESIAN_POINT ( 'NONE',  ( -68.54388738667908854, -279.1383285948262483, -204.2974218086809515 ) ) ;
#43248=CARTESIAN_POINT ( 'NONE',  ( 39.22725684168179328, -276.8030930094064956, -274.0096683686523420 ) ) ;
#43249=CARTESIAN_POINT ( 'NONE',  ( -69.53153403600639137, -299.0451586492719116, -204.1856730493908287 ) ) ;
#43250=CARTESIAN_POINT ( 'NONE',  ( -76.64775181619921796, -282.6230497585922308, -336.3610164745032307 ) ) ;
#43251=CARTESIAN_POINT ( 'NONE',  ( -110.6231407632999719, -292.1760253294439735, -280.8347428600993680 ) ) ;
#43252=CARTESIAN_POINT ( 'NONE',  ( -55.16645527656131520, -275.4267189769729498, -196.2752318955378144 ) ) ;
#43253=CARTESIAN_POINT ( 'NONE',  ( -98.78319446693210182, -298.3690761968088054, -224.5904332186586885 ) ) ;
#43254=CARTESIAN_POINT ( 'NONE',  ( 18.46433878467093237, -296.2481679967467016, -320.2373853464923741 ) ) ;
#43255=CARTESIAN_POINT ( 'NONE',  ( -105.8004833355823990, -282.1552425038193519, -300.5840136956837796 ) ) ;
#43256=CARTESIAN_POINT ( 'NONE',  ( -70.88466519850025804, -291.2883631443361310, -201.0746562027783568 ) ) ;
#43257=CARTESIAN_POINT ( 'NONE',  ( -86.37198171729069429, -271.3881392679651299, -214.0083393153563236 ) ) ;
#43258=CARTESIAN_POINT ( 'NONE',  ( -32.37908468025877795, -287.7138385185117500, -194.3098555151815106 ) ) ;
#43259=CARTESIAN_POINT ( 'NONE',  ( -72.76430206339378515, -290.4919619211961503, -206.1210174028015274 ) ) ;
#43261=CARTESIAN_POINT ( 'NONE',  ( -106.7177755994177062, -289.5411533969804054, -238.2106539605180728 ) ) ;
#43262=CARTESIAN_POINT ( 'NONE',  ( -53.41731125654033008, -288.9308133339569054, -341.5907621872297568 ) ) ;
#43264=CARTESIAN_POINT ( 'NONE',  ( -2.376156507956105557, -287.5834482175696394, -202.0902664909766600 ) ) ;
#43265=CARTESIAN_POINT ( 'NONE',  ( -9.976501702364563684, -277.0180184902516771, -338.0742699716790298 ) ) ;
#43266=CARTESIAN_POINT ( 'NONE',  ( 36.78735426201755843, -292.2248304585155552, -250.6539726117766236 ) ) ;
#43267=CARTESIAN_POINT ( 'NONE',  ( -61.19216622462478483, -284.0051661692461380, -343.5225951486555687 ) ) ;
#43268=CARTESIAN_POINT ( 'NONE',  ( -111.0865003937758360, -284.6077743733175680, -292.4851232668260081 ) ) ;
#43269=CARTESIAN_POINT ( 'NONE',  ( -59.74415356586015946, -280.0872254151739185, -200.8080299144439778 ) ) ;
#43270=CARTESIAN_POINT ( 'NONE',  ( 200.1467820935076247, 289.4019165369547864, -97.55132449765557112 ) ) ;
#43271=CARTESIAN_POINT ( 'NONE',  ( -113.1125314665755326, -270.0723479569915071, -296.1281988589327625 ) ) ;
#43272=CARTESIAN_POINT ( 'NONE',  ( -112.7804352628385942, -270.4057570101002170, -283.7043318166019503 ) ) ;
#43273=CARTESIAN_POINT ( 'NONE',  ( -81.15956189548737143, -272.6368720216149768, -211.7091883079189643 ) ) ;
#43274=CARTESIAN_POINT ( 'NONE',  ( 23.31579562908844849, -273.9021136340691669, -229.1695016566848153 ) ) ;
#43275=CARTESIAN_POINT ( 'NONE',  ( -4.534469127212947370, -294.1390577145843395, -339.9687685013685154 ) ) ;
#43276=CARTESIAN_POINT ( 'NONE',  ( -46.41228527574025264, -155.8298051699933637, -361.8999249830316671 ) ) ;
#43277=CARTESIAN_POINT ( 'NONE',  ( -92.80305917252677261, -271.9620699616363595, -217.6415687889847277 ) ) ;
#43278=CARTESIAN_POINT ( 'NONE',  ( -103.6460653980246605, -298.8594916326841258, -236.8610153399096419 ) ) ;
#43279=CARTESIAN_POINT ( 'NONE',  ( -21.00352826219625868, -290.1532573003599964, -342.0152010249061050 ) ) ;
#43281=CARTESIAN_POINT ( 'NONE',  ( 1.660245709109334111, -295.4851653861246064, -336.4797116896423859 ) ) ;
#43283=CARTESIAN_POINT ( 'NONE',  ( 16.93213062955296877, -287.3445431787742450, -221.4308924556462728 ) ) ;
#43284=CARTESIAN_POINT ( 'NONE',  ( -18.61210145447150310, -273.2081048368760889, -195.9376663295639105 ) ) ;
#43285=CARTESIAN_POINT ( 'NONE',  ( -22.11951685482733865, -295.6647449400144296, -345.6767468812231527 ) ) ;
#43286=CARTESIAN_POINT ( 'NONE',  ( -30.59010156213546949, -295.4612841546360755, -347.0027699742334448 ) ) ;
#43287=CARTESIAN_POINT ( 'NONE',  ( -93.44119962011100711, -291.3817306201440260, -223.6313666735525203 ) ) ;
#43289=CARTESIAN_POINT ( 'NONE',  ( -60.45435088872834939, -275.6750119947716939, -198.3682175567925583 ) ) ;
#43290=CARTESIAN_POINT ( 'NONE',  ( 28.74559755987726817, -274.8539148956148210, -309.0971193516192557 ) ) ;
#43291=ORIENTED_EDGE ( 'NONE', *, *, #23628, .T. ) ;
#43292=CARTESIAN_POINT ( 'NONE',  ( -111.6699499877698543, -278.3093785009016869, -250.4397351406170174 ) ) ;
#43293=CARTESIAN_POINT ( 'NONE',  ( -31.25362233522507793, -272.5301614271577932, -196.7998713559981638 ) ) ;
#43294=CARTESIAN_POINT ( 'NONE',  ( -105.7094784867675372, -273.9855412800620229, -243.7621276016092224 ) ) ;
#43295=CARTESIAN_POINT ( 'NONE',  ( 35.07251602293275283, -276.3485031598098089, -259.3411214982757542 ) ) ;
#43296=CARTESIAN_POINT ( 'NONE',  ( 26.07238527888006274, -276.7544003094457139, -228.4967203951786985 ) ) ;
#43297=CARTESIAN_POINT ( 'NONE',  ( 26.24702249500338880, -274.1149082048291916, -310.8917261157436087 ) ) ;
#43298=CARTESIAN_POINT ( 'NONE',  ( -7.939707988022100871, -295.3079015963584197, -337.3031510345140873 ) ) ;
#43299=CARTESIAN_POINT ( 'NONE',  ( 35.88355451779958116, -292.0247527485320234, -262.5573234989684011 ) ) ;
#43301=CARTESIAN_POINT ( 'NONE',  ( -74.98330416502069795, -280.0569413540614505, -203.2594298606140057 ) ) ;
#43302=CARTESIAN_POINT ( 'NONE',  ( -61.78782538194374041, -277.5454475925818656, -339.1999360838503321 ) ) ;
#43305=CARTESIAN_POINT ( 'NONE',  ( -43.60905962804377367, -284.6595001588505625, -194.0584888816471789 ) ) ;
#43306=CARTESIAN_POINT ( 'NONE',  ( -76.11419864232016153, -297.5686729812242106, -334.8167050964337363 ) ) ;
#43307=CARTESIAN_POINT ( 'NONE',  ( 82.65653505821647684, -298.9546730799231682, -197.7944811758501658 ) ) ;
#43308=CARTESIAN_POINT ( 'NONE',  ( 35.79093094395190633, -286.7942834391931228, -273.7775422583916338 ) ) ;
#43309=CARTESIAN_POINT ( 'NONE',  ( -70.93245602562748786, -275.7415489234395523, -336.3128816752575858 ) ) ;
#43310=CARTESIAN_POINT ( 'NONE',  ( -107.6851990893781732, -276.8408554166956037, -292.1459412301165912 ) ) ;
#43311=CARTESIAN_POINT ( 'NONE',  ( -107.4488627061712549, -286.2044010744293701, -297.1507758768117924 ) ) ;
#43312=CARTESIAN_POINT ( 'NONE',  ( -64.46568126181904290, -278.6191963512717962, -338.6164074463517295 ) ) ;
#43314=CARTESIAN_POINT ( 'NONE',  ( 35.72054554733345810, -274.2269137257707712, -292.0484766116023252 ) ) ;
#43315=CARTESIAN_POINT ( 'NONE',  ( 35.68832738967930851, -276.1477633948825314, -266.1248067559043875 ) ) ;
#43316=CARTESIAN_POINT ( 'NONE',  ( 34.83207928417526489, -283.2820090341699597, -249.3156487456021750 ) ) ;
#43318=CARTESIAN_POINT ( 'NONE',  ( -15.34759292839868472, -290.6899029083019741, -342.7039601795158319 ) ) ;
#43319=CARTESIAN_POINT ( 'NONE',  ( 21.63712020873050790, -290.9157949897243043, -224.0104072398715971 ) ) ;
#43321=CARTESIAN_POINT ( 'NONE',  ( -37.80973136786009547, -296.8410831529566281, -196.9655360109972833 ) ) ;
#43322=CARTESIAN_POINT ( 'NONE',  ( -55.28842110563833501, -289.9584019965592461, -198.3279264411563929 ) ) ;
#43323=CARTESIAN_POINT ( 'NONE',  ( -75.10193482699480683, -210.9688814900462432, -359.8487438039043127 ) ) ;
#43325=CARTESIAN_POINT ( 'NONE',  ( -112.6786424774967941, -288.8789971993604695, -282.4876537846278666 ) ) ;
#43326=CARTESIAN_POINT ( 'NONE',  ( -110.8997504895301063, -282.5497265266225213, -289.4702356246036743 ) ) ;
#43327=CARTESIAN_POINT ( 'NONE',  ( 5.953282685238336924, -283.8771274236851241, -329.8667427487080204 ) ) ;
#43328=CARTESIAN_POINT ( 'NONE',  ( -104.2568765402012048, -284.9577844238124840, -299.9408558479933049 ) ) ;
#43330=CARTESIAN_POINT ( 'NONE',  ( -96.19511238494023075, -293.1761275810710572, -223.3007028383269983 ) ) ;
#43331=CARTESIAN_POINT ( 'NONE',  ( -5.126979291058860966, -274.7979943101187814, -200.4471991034898792 ) ) ;
#43332=CARTESIAN_POINT ( 'NONE',  ( -88.53417205081933616, -287.8433325724970473, -325.9366972801727229 ) ) ;
#43333=CARTESIAN_POINT ( 'NONE',  ( -82.54628190410252842, -277.6509575971571167, -332.6952642144208880 ) ) ;
#43334=CARTESIAN_POINT ( 'NONE',  ( 29.88666486062728822, -295.9627297293893662, -302.9179393708922134 ) ) ;
#43337=CARTESIAN_POINT ( 'NONE',  ( -103.4636256423404319, -282.8042152529550890, -302.5581743686024652 ) ) ;
#43338=CARTESIAN_POINT ( 'NONE',  ( -45.04201984405015935, -277.9546122620739652, -195.7058468397716240 ) ) ;
#43339=CARTESIAN_POINT ( 'NONE',  ( -76.06404202801982706, -272.0249580168496095, -204.5483572420409644 ) ) ;
#43340=CARTESIAN_POINT ( 'NONE',  ( 18.38073660658709585, -275.5726126801830560, -317.6781626157851974 ) ) ;
#43341=CARTESIAN_POINT ( 'NONE',  ( 35.39518030445368879, -294.9166019605768270, -258.4478949576399600 ) ) ;
#43342=CARTESIAN_POINT ( 'NONE',  ( -9.649584533061148051, -293.3641616281943243, -202.5092646401708407 ) ) ;
#43343=CARTESIAN_POINT ( 'NONE',  ( 38.94805206123166386, -294.7948292798829470, -264.6016056227712738 ) ) ;
#43344=CARTESIAN_POINT ( 'NONE',  ( -108.4765597226606531, -296.6017643412727125, -253.9650283572826766 ) ) ;
#43345=CARTESIAN_POINT ( 'NONE',  ( -40.00409389572237728, -291.0856444169626229, -345.3647856263623339 ) ) ;
#43346=CARTESIAN_POINT ( 'NONE',  ( -30.21277951589942035, -283.1309896249060785, -347.0303979805375434 ) ) ;
#43347=CARTESIAN_POINT ( 'NONE',  ( 8.777517695267203379, -272.8165299731578557, -210.2501936411803456 ) ) ;
#43348=CARTESIAN_POINT ( 'NONE',  ( 38.10786404863083732, -287.5777474754362402, -285.7352283656842928 ) ) ;
#43349=CARTESIAN_POINT ( 'NONE',  ( -96.56291439218715311, -279.9068103850914326, -315.8000284812546852 ) ) ;
#43351=CARTESIAN_POINT ( 'NONE',  ( -22.40015596388471764, -285.3067938223641136, -198.6141681104379302 ) ) ;
#43352=CARTESIAN_POINT ( 'NONE',  ( -104.7280414750854192, -288.1165675280980736, -303.4046435690154340 ) ) ;
#43353=CARTESIAN_POINT ( 'NONE',  ( -115.8664652629750549, -267.0802710791712116, -295.7299871733738996 ) ) ;
#43354=CARTESIAN_POINT ( 'NONE',  ( -108.7815577518589265, -283.8572520999057360, -285.7285719363633234 ) ) ;
#43355=CARTESIAN_POINT ( 'NONE',  ( 24.26322914733271929, -282.1490045742972370, -224.8326498721849021 ) ) ;
#43356=CARTESIAN_POINT ( 'NONE',  ( -107.5211435740363868, -289.2112476431066170, -301.5992326614872354 ) ) ;
#43357=CARTESIAN_POINT ( 'NONE',  ( -45.21123133330947752, -281.5543207393445186, -194.5161261155256796 ) ) ;
#43358=CARTESIAN_POINT ( 'NONE',  ( -61.90525397699875754, -281.0547061122641708, -197.8488397926061850 ) ) ;
#43359=CARTESIAN_POINT ( 'NONE',  ( -34.31120346350135719, -279.9245943571611406, -197.4115050792045736 ) ) ;
#43360=CARTESIAN_POINT ( 'NONE',  ( -8.354870553190677285, -276.4132869994372186, -201.5192985566135917 ) ) ;
#43361=CARTESIAN_POINT ( 'NONE',  ( 39.50214713631897467, -293.6231637474240301, -276.0391462781040559 ) ) ;
#43362=CARTESIAN_POINT ( 'NONE',  ( -40.04234839696056270, -287.1062376042696656, -345.0077492016332599 ) ) ;
#43363=CARTESIAN_POINT ( 'NONE',  ( -40.61862575140684584, -293.6117397404952385, -194.2185636389559136 ) ) ;
#43364=CARTESIAN_POINT ( 'NONE',  ( -96.66662287155928368, -294.8720686276568017, -313.4497018574463141 ) ) ;
#43365=CARTESIAN_POINT ( 'NONE',  ( -37.51988987875960646, -284.9745879434625522, -344.8135828466392923 ) ) ;
#43366=CARTESIAN_POINT ( 'NONE',  ( -55.81275597118737863, -294.9631699522789745, -341.0598731621005300 ) ) ;
#43367=CARTESIAN_POINT ( 'NONE',  ( -86.32620317555371514, -292.4705895245837155, -211.2835870222715187 ) ) ;
#43368=CARTESIAN_POINT ( 'NONE',  ( 33.20978049366844687, -281.9504969847442908, -251.1721590282433567 ) ) ;
#43369=CARTESIAN_POINT ( 'NONE',  ( -107.8566035761110129, -272.0000889936525823, -239.8875109574228759 ) ) ;
#43370=CARTESIAN_POINT ( 'NONE',  ( -69.30735587525889230, -290.1131813351529445, -340.3148499007525629 ) ) ;
#43371=CARTESIAN_POINT ( 'NONE',  ( -37.33847804324527431, -281.1916664934377650, -346.1387768952744750 ) ) ;
#43372=CARTESIAN_POINT ( 'NONE',  ( -99.19013785467485889, -291.4951141064793774, -224.5076586840816617 ) ) ;
#43373=CARTESIAN_POINT ( 'NONE',  ( 19.52898507467300249, -287.2378303648362703, -224.5394234360309724 ) ) ;
#43375=CARTESIAN_POINT ( 'NONE',  ( -78.93342798129256721, -207.3472289075424726, -354.9948781244794986 ) ) ;
#43376=CARTESIAN_POINT ( 'NONE',  ( -62.72819003750708333, -182.7653398274297842, -358.6004343349099486 ) ) ;
#43377=CARTESIAN_POINT ( 'NONE',  ( -99.31730995789541794, -277.2124897904703289, -309.3353976584218117 ) ) ;
#43378=CARTESIAN_POINT ( 'NONE',  ( -81.46300260621561051, -278.3565017537416111, -211.7522160558771986 ) ) ;
#43379=CARTESIAN_POINT ( 'NONE',  ( -38.35287593860172706, -273.7065218918179994, -193.3889034170015861 ) ) ;
#43380=CARTESIAN_POINT ( 'NONE',  ( -87.43554566246351101, -230.9673987827994210, -345.9252775359201451 ) ) ;
#43381=CARTESIAN_POINT ( 'NONE',  ( -99.75712166490203003, -277.7146594378781970, -226.2825353398110906 ) ) ;
#43382=CARTESIAN_POINT ( 'NONE',  ( -40.32477459187423108, -281.1099505302134958, -344.9462912529492087 ) ) ;
#43383=CARTESIAN_POINT ( 'NONE',  ( -110.2368565160181078, -298.0390585385410418, -291.8608737959810924 ) ) ;
#43384=CARTESIAN_POINT ( 'NONE',  ( -0.06494025528746319442, -293.0551079096751437, -207.5245711721255759 ) ) ;
#43385=CARTESIAN_POINT ( 'NONE',  ( -13.14117805953388007, -287.4158688506900035, -339.7554852554226841 ) ) ;
#43386=CARTESIAN_POINT ( 'NONE',  ( -32.69705956757077558, -274.7606237578257833, -193.5903134513877148 ) ) ;
#43387=CARTESIAN_POINT ( 'NONE',  ( -92.01815984315234687, -273.2432029712903727, -221.9928974961060817 ) ) ;
#43391=CARTESIAN_POINT ( 'NONE',  ( -102.1885730148448630, -280.9888025511481828, -231.4753474475529913 ) ) ;
#43392=CARTESIAN_POINT ( 'NONE',  ( -16.84842264494902508, -281.4028238013963232, -199.9746729037055104 ) ) ;
#43393=CARTESIAN_POINT ( 'NONE',  ( -22.78258808288043369, -281.9959965722508173, -195.7287196729666050 ) ) ;
#43394=CARTESIAN_POINT ( 'NONE',  ( -61.62400858236756562, -282.4341501583178342, -339.5070612325035313 ) ) ;
#43395=CARTESIAN_POINT ( 'NONE',  ( -98.65590310181080724, -279.8399778066235513, -312.2112553115475180 ) ) ;
#43396=CARTESIAN_POINT ( 'NONE',  ( -16.42551273587970684, -272.8071510119688696, -199.6451780863918657 ) ) ;
#43399=CARTESIAN_POINT ( 'NONE',  ( 34.56703283253786196, -276.0116629786900262, -243.2817357121049042 ) ) ;
#43401=CARTESIAN_POINT ( 'NONE',  ( 23.68432002420183835, -276.9591021982989218, -226.7406999239534571 ) ) ;
#43402=CARTESIAN_POINT ( 'NONE',  ( -54.02045038036295210, -275.8368251194293066, -344.9836039973096717 ) ) ;
#43403=VERTEX_POINT ( 'NONE', #43893 ) ;
#43405=CARTESIAN_POINT ( 'NONE',  ( -105.5068348888408281, -286.1115707025226129, -302.4846483425838528 ) ) ;
#43407=CARTESIAN_POINT ( 'NONE',  ( 13.02170408912212274, -291.9749491666452741, -217.2939036000848887 ) ) ;
#43408=CARTESIAN_POINT ( 'NONE',  ( -10.02240465606981523, -285.7481026732858140, -198.4227586823534466 ) ) ;
#43409=CARTESIAN_POINT ( 'NONE',  ( -91.49800515898722608, -282.0765132019558337, -320.8097912973016719 ) ) ;
#43410=CARTESIAN_POINT ( 'NONE',  ( -99.53868827011000064, -282.5866061869135706, -309.7873220949351207 ) ) ;
#43411=CARTESIAN_POINT ( 'NONE',  ( 18.87950669965240280, -284.9499527188662569, -221.5708515069829616 ) ) ;
#43412=CARTESIAN_POINT ( 'NONE',  ( -48.37330104161164712, -284.4007774608808745, -342.9244302366724924 ) ) ;
#43413=CARTESIAN_POINT ( 'NONE',  ( -65.45331386515763938, -271.6845087390630056, -200.8150391709323799 ) ) ;
#43414=CARTESIAN_POINT ( 'NONE',  ( -99.15163841191592553, -282.3539584491877577, -315.0135724021374699 ) ) ;
#43415=CARTESIAN_POINT ( 'NONE',  ( -111.2289657237812435, -298.3832841288626696, -283.5254160638536973 ) ) ;
#43416=CARTESIAN_POINT ( 'NONE',  ( -62.56175086624408976, -283.7245651211972586, -199.5516732280953534 ) ) ;
#43417=CARTESIAN_POINT ( 'NONE',  ( -109.3656735607848987, -279.6678302470750737, -257.0962885614056290 ) ) ;
#43418=CARTESIAN_POINT ( 'NONE',  ( 37.74472285456480591, -289.4951776745472785, -265.9011675192144253 ) ) ;
#43421=CARTESIAN_POINT ( 'NONE',  ( 18.48263136099120274, -296.1784363810049854, -321.3584557497873107 ) ) ;
#43422=CARTESIAN_POINT ( 'NONE',  ( -88.47725723244910512, -275.7689532948882629, -325.2260015257643886 ) ) ;
#43423=CARTESIAN_POINT ( 'NONE',  ( -99.74511591218792717, -289.1535987420851370, -315.2163816133560772 ) ) ;
#43424=CARTESIAN_POINT ( 'NONE',  ( -28.82365413389263864, -293.3423726761366197, -343.7194648805318593 ) ) ;
#43425=CARTESIAN_POINT ( 'NONE',  ( -106.9061215607682271, -277.5517736839869940, -246.4976734086177999 ) ) ;
#43426=CARTESIAN_POINT ( 'NONE',  ( -93.08048571575984909, -271.3233591039005432, -221.0204453008902590 ) ) ;
#43427=CARTESIAN_POINT ( 'NONE',  ( -17.31418827951640793, -293.6311327765207579, -199.5964903536095392 ) ) ;
#43428=CARTESIAN_POINT ( 'NONE',  ( -54.49178911615188525, -282.3376638359844719, -195.3683826091709363 ) ) ;
#43429=CARTESIAN_POINT ( 'NONE',  ( 20.82645875388856282, -292.7038562863409652, -319.7491028241295794 ) ) ;
#43430=CARTESIAN_POINT ( 'NONE',  ( -64.09207112628276093, -291.0070040632829205, -339.1971234759729441 ) ) ;
#43431=CARTESIAN_POINT ( 'NONE',  ( -97.37302182073817391, -288.1616190127863888, -316.9466783307221931 ) ) ;
#43432=CARTESIAN_POINT ( 'NONE',  ( 29.97132445528106359, -289.3759147627188213, -300.2253297965915522 ) ) ;
#43434=CARTESIAN_POINT ( 'NONE',  ( -75.94528405702773455, -290.3850811402107297, -332.5090466261805773 ) ) ;
#43435=EDGE_CURVE ( 'NONE', #93199, #38700, #77682, .T. ) ;
#43437=CARTESIAN_POINT ( 'NONE',  ( -5.776024410489380756, -289.8513142760285177, -340.1580866586363072 ) ) ;
#43438=CARTESIAN_POINT ( 'NONE',  ( -47.86363211020864128, -277.9392164427554803, -195.6914320520579338 ) ) ;
#43439=CARTESIAN_POINT ( 'NONE',  ( -67.35812943433514022, -280.0023844680056300, -199.4755886886987355 ) ) ;
#43440=CARTESIAN_POINT ( 'NONE',  ( 26.70193986459174695, -281.7812112698554756, -313.0712627727609174 ) ) ;
#43441=CARTESIAN_POINT ( 'NONE',  ( 12.48118591435941482, -284.7456518849382974, -214.2317021613211807 ) ) ;
#43443=CARTESIAN_POINT ( 'NONE',  ( -5.524678771183688220, -280.7687758078539559, -337.4462752216025478 ) ) ;
#43444=CARTESIAN_POINT ( 'NONE',  ( -110.5777956472695536, -282.3443717226074341, -286.5313055646341809 ) ) ;
#43446=CARTESIAN_POINT ( 'NONE',  ( -99.10011729990263518, -276.4317910522534589, -315.2008141437713107 ) ) ;
#43447=CARTESIAN_POINT ( 'NONE',  ( -105.1523238591232428, -283.9381583100451394, -234.4255049019193962 ) ) ;
#43448=CARTESIAN_POINT ( 'NONE',  ( 9.104247122874012277, -299.5888637825325418, -197.1181713360114713 ) ) ;
#43449=CARTESIAN_POINT ( 'NONE',  ( -107.3364329621977049, -292.4595799038322070, -246.9692862814247860 ) ) ;
#43450=CARTESIAN_POINT ( 'NONE',  ( -44.00956919143204971, -275.3948251415978348, -194.1889303908548072 ) ) ;
#43451=CARTESIAN_POINT ( 'NONE',  ( 35.12652270509740760, -275.3424674864635335, -279.7332566004096179 ) ) ;
#43452=CARTESIAN_POINT ( 'NONE',  ( -87.81770607290447117, -297.7577978263153113, -325.8333945734870554 ) ) ;
#43453=CARTESIAN_POINT ( 'NONE',  ( 5.559083387748535721, -288.6550865633099647, -334.3026755036227655 ) ) ;
#43454=CARTESIAN_POINT ( 'NONE',  ( 37.97827302712818209, -279.5553000099262704, -264.3431582021373174 ) ) ;
#43455=CARTESIAN_POINT ( 'NONE',  ( -4.602216920455489912, -292.3049943157915891, -200.6680319278289915 ) ) ;
#43456=EDGE_CURVE ( 'NONE', #34721, #92061, #57163, .T. ) ;
#43457=CARTESIAN_POINT ( 'NONE',  ( -109.5065327083319744, -289.7787481143462287, -257.5960518501238425 ) ) ;
#43458=CARTESIAN_POINT ( 'NONE',  ( -17.07252644415595810, -292.7904386113723945, -342.6240595373823226 ) ) ;
#43461=CARTESIAN_POINT ( 'NONE',  ( 30.88809663704017439, -292.7111455752344114, -244.2329095684307276 ) ) ;
#43463=CARTESIAN_POINT ( 'NONE',  ( -3.603613472001642393, -287.4277866820104350, -201.3933057632786472 ) ) ;
#43464=CARTESIAN_POINT ( 'NONE',  ( -92.08974858914540107, -275.4094976428775681, -313.9805196606274080 ) ) ;
#43465=CARTESIAN_POINT ( 'NONE',  ( -56.02465264753779195, -294.3458410997327519, -344.8175985429817842 ) ) ;
#43466=CARTESIAN_POINT ( 'NONE',  ( -97.20506964720831888, -286.5092331376041557, -222.7200090002236266 ) ) ;
#43467=CARTESIAN_POINT ( 'NONE',  ( -109.6119255445987193, -284.5212970642943446, -260.0647825785431451 ) ) ;
#43468=CARTESIAN_POINT ( 'NONE',  ( 32.71494593002077522, -276.7697930191113755, -247.3328422661348043 ) ) ;
#43469=CARTESIAN_POINT ( 'NONE',  ( 0.04449511879383971635, -292.5724611573358516, -335.0275253664256638 ) ) ;
#43470=CARTESIAN_POINT ( 'NONE',  ( 34.43417773083176314, -295.5473916441992515, -288.4220529946449005 ) ) ;
#43471=CARTESIAN_POINT ( 'NONE',  ( -26.98054600509038181, -275.7123912716060659, -343.0231919231287634 ) ) ;
#43474=CARTESIAN_POINT ( 'NONE',  ( -50.46809359016861407, -294.8819516350542926, -346.2664960106724266 ) ) ;
#43475=CARTESIAN_POINT ( 'NONE',  ( 33.69501238127471510, -289.7635006161941646, -292.7836949668480315 ) ) ;
#43477=CARTESIAN_POINT ( 'NONE',  ( -48.93688340976666495, -298.9875598468339035, -194.4984038835194156 ) ) ;
#43479=CARTESIAN_POINT ( 'NONE',  ( -14.54207697897043872, -287.0069175899264451, -200.8525035688566902 ) ) ;
#43481=CARTESIAN_POINT ( 'NONE',  ( -99.23104185823777357, -278.2161651401011682, -224.9238565318159431 ) ) ;
#43482=CARTESIAN_POINT ( 'NONE',  ( -0.7473656586055850148, -295.2306030980432183, -338.0085760740752789 ) ) ;
#43483=CARTESIAN_POINT ( 'NONE',  ( -10.03103973441768026, -286.8389096837565830, -341.0324226925332027 ) ) ;
#43484=CARTESIAN_POINT ( 'NONE',  ( -88.58819105861471144, -296.0809220854289379, -327.8742298937423243 ) ) ;
#43485=CARTESIAN_POINT ( 'NONE',  ( 35.31591808069838834, -293.7830228634124410, -262.5954492359664414 ) ) ;
#43488=CARTESIAN_POINT ( 'NONE',  ( -82.08642841125383427, -219.1949203529638623, -349.1242040296363598 ) ) ;
#43489=CARTESIAN_POINT ( 'NONE',  ( -35.18738530977717005, -287.5988232182348270, -194.0718402913028910 ) ) ;
#43490=CARTESIAN_POINT ( 'NONE',  ( -88.52914483777347243, -293.1952119285919025, -334.4957818155094174 ) ) ;
#43492=CARTESIAN_POINT ( 'NONE',  ( -107.3229105242246106, -278.3101404745816012, -238.3590844367061266 ) ) ;
#43493=CARTESIAN_POINT ( 'NONE',  ( -56.77095638343554640, -285.3034222921888841, -342.6282088674892066 ) ) ;
#43494=CARTESIAN_POINT ( 'NONE',  ( -70.79178560055378000, -284.1942628544149443, -201.6610591947422222 ) ) ;
#43495=CARTESIAN_POINT ( 'NONE',  ( -5.192225229086207428, -286.7055107458209591, -337.5007148370161758 ) ) ;
#43496=CARTESIAN_POINT ( 'NONE',  ( -8.335256994194917723, -278.5368422520412537, -340.3675447722445142 ) ) ;
#43497=CARTESIAN_POINT ( 'NONE',  ( -72.88229652963883609, -298.0599882713836450, -206.5265313608019540 ) ) ;
#43499=CARTESIAN_POINT ( 'NONE',  ( 34.25204703431068509, -292.4551521410048736, -287.0170711653544231 ) ) ;
#43500=CARTESIAN_POINT ( 'NONE',  ( -104.2713891148673895, -278.1587637744920016, -299.6325371492179670 ) ) ;
#43501=CARTESIAN_POINT ( 'NONE',  ( -81.34262857331447094, -278.7846910316441154, -211.9211021829239030 ) ) ;
#43502=CARTESIAN_POINT ( 'NONE',  ( 38.42008636018527312, -276.4813143978914809, -258.3751275733171155 ) ) ;
#43503=CARTESIAN_POINT ( 'NONE',  ( -45.62993176495204750, -276.0750550011469500, -346.6556697337338164 ) ) ;
#43504=CARTESIAN_POINT ( 'NONE',  ( -23.51153694099567915, -107.8100564029413704, -360.1567311266264824 ) ) ;
#43505=CARTESIAN_POINT ( 'NONE',  ( -108.8794380750494213, -297.6334543093705634, -297.3609688603785344 ) ) ;
#43506=CARTESIAN_POINT ( 'NONE',  ( -37.37352853689063892, -276.5519495502701943, -195.3611179825600175 ) ) ;
#43509=CARTESIAN_POINT ( 'NONE',  ( -38.64413161842912814, -287.1151491696821836, -197.0510410699282886 ) ) ;
#43510=CARTESIAN_POINT ( 'NONE',  ( -10.37482758168705388, -288.1592681364655846, -199.2645073152849875 ) ) ;
#43511=CARTESIAN_POINT ( 'NONE',  ( -31.87199579458728493, -288.3300365010234714, -343.3088282413960997 ) ) ;
#43512=CARTESIAN_POINT ( 'NONE',  ( -44.41980399959960835, -282.6469378582092986, -347.0266209547609151 ) ) ;
#43513=CARTESIAN_POINT ( 'NONE',  ( -105.1694075032272764, -277.3384911008652125, -241.2777460070076643 ) ) ;
#43514=CARTESIAN_POINT ( 'NONE',  ( -111.6262676631040165, -286.4050373414812043, -270.9422197182587411 ) ) ;
#43515=CARTESIAN_POINT ( 'NONE',  ( -57.28240059536676654, -278.2699859010681962, -199.4169412261406649 ) ) ;
#43516=CARTESIAN_POINT ( 'NONE',  ( -89.42355889430436378, -279.1195276500897648, -322.2862689286160389 ) ) ;
#43517=CARTESIAN_POINT ( 'NONE',  ( 11.58308369440831953, -275.2450472520770859, -216.0311002410117283 ) ) ;
#43518=CARTESIAN_POINT ( 'NONE',  ( -51.62638300111430567, -288.0259101326500968, -345.6203802214030816 ) ) ;
#43519=CARTESIAN_POINT ( 'NONE',  ( -5.513057092220508437, -283.4468357167801287, -340.2974912342566540 ) ) ;
#43520=CARTESIAN_POINT ( 'NONE',  ( -47.24222819239442117, -283.6670915203624190, -346.6599151367047966 ) ) ;
#43521=EDGE_LOOP ( 'NONE', ( #93558, #21920 ) ) ;
#43523=DIRECTION ( 'NONE',  ( 0.000000000000000000, 0.000000000000000000, -1.000000000000000000 ) ) ;
#43524=CARTESIAN_POINT ( 'NONE',  ( -29.08781290339920389, -290.8091620183986947, -345.7276551782750289 ) ) ;
#43525=CARTESIAN_POINT ( 'NONE',  ( -101.8942289069071734, -288.6941554437736386, -311.5228501339166201 ) ) ;
#43527=CARTESIAN_POINT ( 'NONE',  ( -59.53557361278180338, -272.8164568751031425, -200.5166226242758398 ) ) ;
#43528=CARTESIAN_POINT ( 'NONE',  ( 39.60962277385706187, -292.9002039593197537, -270.3183063866856628 ) ) ;
#43529=CARTESIAN_POINT ( 'NONE',  ( -58.91037137977332350, -287.8160346317469021, -340.8807337726425999 ) ) ;
#43530=CARTESIAN_POINT ( 'NONE',  ( 0.4454132180781383843, -290.8029828628548898, -206.7206585370008156 ) ) ;
#43531=CARTESIAN_POINT ( 'NONE',  ( 26.04667951827650185, -289.2635271134293475, -307.4622218789428985 ) ) ;
#43532=CARTESIAN_POINT ( 'NONE',  ( 21.31550574532285580, -290.6948066931273615, -317.0979686699210447 ) ) ;
#43533=CARTESIAN_POINT ( 'NONE',  ( 19.97742372891767815, -290.2212647443581091, -318.7296893090459093 ) ) ;
#43534=CARTESIAN_POINT ( 'NONE',  ( -58.40006995558686498, -289.7803841335240804, -198.2045279563109830 ) ) ;
#43535=CARTESIAN_POINT ( 'NONE',  ( -76.66686770079212465, -293.5264245113584138, -206.4381724166781567 ) ) ;
#43536=CARTESIAN_POINT ( 'NONE',  ( -108.3183126739273661, -285.2559594128039180, -288.4090796484070438 ) ) ;
#43537=CARTESIAN_POINT ( 'NONE',  ( -47.52094747803085539, -293.9233500542866864, -195.8343694083687296 ) ) ;
#43538=CARTESIAN_POINT ( 'NONE',  ( -113.3425974752031493, -270.8076308035728061, -270.3389060467516174 ) ) ;
#43539=CARTESIAN_POINT ( 'NONE',  ( -15.35796352212545912, -300.2454598573677345, -194.7939833255516078 ) ) ;
#43540=CARTESIAN_POINT ( 'NONE',  ( 35.84916290400889238, -280.7260000434499716, -268.5898457665853130 ) ) ;
#43541=CARTESIAN_POINT ( 'NONE',  ( -84.05991212271342761, -281.6935959886387195, -329.0998267559237433 ) ) ;
#43542=CARTESIAN_POINT ( 'NONE',  ( -50.45005498846544612, -294.4124758169335792, -346.1271020356829240 ) ) ;
#43543=CARTESIAN_POINT ( 'NONE',  ( 22.31101732609832666, -273.1866000526096627, -226.5487074624397792 ) ) ;
#43544=CARTESIAN_POINT ( 'NONE',  ( -111.7905492138154671, -276.6646643336296165, -267.8354834178849728 ) ) ;
#43545=CARTESIAN_POINT ( 'NONE',  ( -68.27022746863505631, -298.9523956380553500, -203.6790041995958518 ) ) ;
#43546=CARTESIAN_POINT ( 'NONE',  ( -34.10981224036434156, -272.6667863161680430, -194.0187235045170553 ) ) ;
#43547=CARTESIAN_POINT ( 'NONE',  ( 34.52131233576097458, -294.7693090364884370, -254.4573361343793181 ) ) ;
#43549=CARTESIAN_POINT ( 'NONE',  ( 19.82633579470533647, -294.9986640864898959, -316.0365131792631814 ) ) ;
#43551=CARTESIAN_POINT ( 'NONE',  ( -29.60616973671221785, -284.1697682403773797, -195.4040077689209056 ) ) ;
#43552=CARTESIAN_POINT ( 'NONE',  ( -103.9366167652389095, -296.1478869058889813, -300.3864741894257691 ) ) ;
#43553=CARTESIAN_POINT ( 'NONE',  ( -109.0284809337596101, -284.9100685495209859, -242.1090782600143427 ) ) ;
#43554=CARTESIAN_POINT ( 'NONE',  ( 23.84721203567875847, -286.5957326044330671, -223.6312468062063203 ) ) ;
#43555=CARTESIAN_POINT ( 'NONE',  ( 0.8664747166047355176, -290.5630023237768569, -206.0170133456105930 ) ) ;
#43556=CARTESIAN_POINT ( 'NONE',  ( -101.7502699662694994, -278.3018715467194397, -228.3638444514133141 ) ) ;
#43557=CARTESIAN_POINT ( 'NONE',  ( 10.64812456238590599, -278.1952119285918457, -210.2361428286349394 ) ) ;
#43559=CARTESIAN_POINT ( 'NONE',  ( 35.95014289420876707, -286.2842879673328866, -265.5760246650050362 ) ) ;
#43560=CARTESIAN_POINT ( 'NONE',  ( -82.68101052597201317, -288.5761969922439789, -332.2144884773866238 ) ) ;
#43563=CARTESIAN_POINT ( 'NONE',  ( -100.8445759073984647, -297.6400093711162071, -308.0625622008096229 ) ) ;
#43564=CARTESIAN_POINT ( 'NONE',  ( -56.42716089895206721, -281.2362843987488645, -196.3176743493169738 ) ) ;
#43565=CARTESIAN_POINT ( 'NONE',  ( -104.5034437540514887, -294.1213101860024040, -304.6478662851592958 ) ) ;
#43566=CARTESIAN_POINT ( 'NONE',  ( 31.99802314604900744, -280.9131540185737208, -247.3087051468501443 ) ) ;
#43567=CARTESIAN_POINT ( 'NONE',  ( 1.771263359367746260, -294.7107183991899433, -336.6874030566929150 ) ) ;
#43568=CARTESIAN_POINT ( 'NONE',  ( 11.17209960989293727, -284.7974003236965359, -212.3642015460783625 ) ) ;
#43569=CARTESIAN_POINT ( 'NONE',  ( -70.37720994900570304, -281.6168532604185089, -203.0286908453328749 ) ) ;
#43570=CARTESIAN_POINT ( 'NONE',  ( -106.9266027588686683, -295.9148765568199337, -247.3673440217181962 ) ) ;
#43573=CARTESIAN_POINT ( 'NONE',  ( -83.79914694217985982, -285.6730082613418062, -328.8530403068154442 ) ) ;
#43575=CARTESIAN_POINT ( 'NONE',  ( -37.30987171927208834, -289.5523547857347353, -195.3611179825600175 ) ) ;
#43576=CARTESIAN_POINT ( 'NONE',  ( 8.137242795908855797, -275.6453080563344429, -332.3610216312295620 ) ) ;
#43577=CARTESIAN_POINT ( 'NONE',  ( -107.7513244488335573, -290.6401191635279702, -251.0871768305287901 ) ) ;
#43578=CARTESIAN_POINT ( 'NONE',  ( 26.16627646168965882, -283.5820830503559478, -307.8444095038620958 ) ) ;
#43579=CARTESIAN_POINT ( 'NONE',  ( -49.02192600409640022, -275.5011472350892632, -197.4395479601549539 ) ) ;
#43580=CARTESIAN_POINT ( 'NONE',  ( 8.741356655557691369, -284.0322707069191779, -331.0471319471915308 ) ) ;
#43581=CARTESIAN_POINT ( 'NONE',  ( 20.48437603630994275, -280.9807989981646301, -315.5637221284270026 ) ) ;
#43582=CARTESIAN_POINT ( 'NONE',  ( -108.3462206651810789, -280.8665737772173543, -246.0486506677223701 ) ) ;
#43583=CARTESIAN_POINT ( 'NONE',  ( -108.0783415563494714, -273.1078427050683217, -239.8070697769145454 ) ) ;
#43584=CARTESIAN_POINT ( 'NONE',  ( 16.02856474352110183, -274.6173854097442586, -214.8578313048464281 ) ) ;
#43585=CARTESIAN_POINT ( 'NONE',  ( 31.17170886458801959, -295.0875115833463269, -241.1221824460717755 ) ) ;
#43589=CARTESIAN_POINT ( 'NONE',  ( -2.556030035352807150, -292.7365998118771131, -337.6683437417710252 ) ) ;
#43591=CARTESIAN_POINT ( 'NONE',  ( -6.497303379122718603, -273.9761888997055053, -204.1296176895979784 ) ) ;
#43592=CARTESIAN_POINT ( 'NONE',  ( -70.61305118522868440, -293.1414661854296924, -201.6899817264562387 ) ) ;
#43593=CARTESIAN_POINT ( 'NONE',  ( -37.37352853689063892, -276.5519495502701943, -195.3611179825600175 ) ) ;
#43594=CARTESIAN_POINT ( 'NONE',  ( -2.251474464674564580, -293.7111353148000035, -202.2532112226196830 ) ) ;
#43595=CARTESIAN_POINT ( 'NONE',  ( -26.17682149680866743, -290.9099957426690821, -344.4092206530166891 ) ) ;
#43596=CARTESIAN_POINT ( 'NONE',  ( -86.32402219903653418, -275.7331791068950224, -327.0050453120750831 ) ) ;
#43597=CARTESIAN_POINT ( 'NONE',  ( -92.00906063858325012, -279.7599515512611674, -320.9612480495015916 ) ) ;
#43598=CARTESIAN_POINT ( 'NONE',  ( 36.33643088854014991, -291.4945711850214707, -259.7381613320289944 ) ) ;
#43599=CARTESIAN_POINT ( 'NONE',  ( 22.44309122558506076, -284.0446433533261370, -316.9233007567825666 ) ) ;
#43601=CARTESIAN_POINT ( 'NONE',  ( -29.44658400780438967, -282.6162521331363564, -343.0047117862945925 ) ) ;
#43602=CARTESIAN_POINT ( 'NONE',  ( -19.84018028442471504, -281.3515772202551375, -195.6393795387294574 ) ) ;
#43603=CARTESIAN_POINT ( 'NONE',  ( -92.16035567197184264, -282.6093419098990580, -323.8674140848385719 ) ) ;
#43604=CARTESIAN_POINT ( 'NONE',  ( -111.9436626716666723, -279.2657329460377014, -288.5094373461789132 ) ) ;
#43606=CARTESIAN_POINT ( 'NONE',  ( 34.06606036054898823, -276.7288368117229993, -243.4605697820171315 ) ) ;
#43607=CARTESIAN_POINT ( 'NONE',  ( -53.28691492658256834, -285.7662352645559736, -340.3683826091709079 ) ) ;
#43609=CARTESIAN_POINT ( 'NONE',  ( -111.7104903519865076, -274.6594503043100985, -262.0357671750476811 ) ) ;
#43610=CARTESIAN_POINT ( 'NONE',  ( -106.8074949376054690, -276.2149762292806372, -297.6805277849293248 ) ) ;
#43611=CARTESIAN_POINT ( 'NONE',  ( -71.73393836630971521, -293.3641723441973568, -202.5886988391316663 ) ) ;
#43612=CARTESIAN_POINT ( 'NONE',  ( 20.59892986062730813, -293.5274092912360402, -314.9548765204012284 ) ) ;
#43613=CARTESIAN_POINT ( 'NONE',  ( -105.1047351766068800, -289.5883302215836466, -306.7987082442656401 ) ) ;
#43615=CARTESIAN_POINT ( 'NONE',  ( 39.01738692413017162, -292.1622951732381921, -273.1711208145893011 ) ) ;
#43616=CARTESIAN_POINT ( 'NONE',  ( -102.9402803234467711, -283.4067058632400062, -236.5488910603832551 ) ) ;
#43617=CARTESIAN_POINT ( 'NONE',  ( -99.34403851998186497, -292.9703891159703062, -229.4439881997940347 ) ) ;
#43618=CARTESIAN_POINT ( 'NONE',  ( -5.806240482724225771, -283.9438512781578652, -336.7583809588232953 ) ) ;
#43619=CARTESIAN_POINT ( 'NONE',  ( -111.6911374074538088, -291.2529879756687592, -289.5181570182043629 ) ) ;
#43620=CARTESIAN_POINT ( 'NONE',  ( -35.66767023911081225, -280.5660321961086652, -197.3063466177145244 ) ) ;
#43621=CARTESIAN_POINT ( 'NONE',  ( 37.93788804169939510, -292.1688570614683158, -256.1839418016618311 ) ) ;
#43622=CARTESIAN_POINT ( 'NONE',  ( 30.22558105768289138, -288.8305560230214155, -307.0623292242091793 ) ) ;
#43623=CARTESIAN_POINT ( 'NONE',  ( -5.646114155181704675, -289.1387010115369662, -340.4675851114491252 ) ) ;
#43624=CARTESIAN_POINT ( 'NONE',  ( -17.17391338219007935, -286.4863944786068828, -200.1494481451148886 ) ) ;
#43627=CARTESIAN_POINT ( 'NONE',  ( 38.41994344512264092, -295.3756935967861637, -267.4598827907016698 ) ) ;
#43628=CARTESIAN_POINT ( 'NONE',  ( -113.8733620336338532, -295.2108179121724447, -272.4395755413561346 ) ) ;
#43629=CARTESIAN_POINT ( 'NONE',  ( -110.1392859604227539, -277.4998633469374454, -278.8050807163190257 ) ) ;
#43630=CARTESIAN_POINT ( 'NONE',  ( -114.2801616667020426, -272.0598842126317436, -270.3548630465568863 ) ) ;
#43631=CARTESIAN_POINT ( 'NONE',  ( -37.01170354081605751, -293.5277905846670023, -344.0662568071866190 ) ) ;
#43632=CARTESIAN_POINT ( 'NONE',  ( 21.65808797953431863, -277.9316511720170411, -315.0489129504841230 ) ) ;
#43633=CARTESIAN_POINT ( 'NONE',  ( -111.1106114664330136, -270.7994961627850898, -262.0536996530543092 ) ) ;
#43634=CARTESIAN_POINT ( 'NONE',  ( 30.21524673366255342, -294.3725483484116694, -241.5398772946525980 ) ) ;
#43635=CARTESIAN_POINT ( 'NONE',  ( -66.16205118845314814, -296.5181744713414105, -337.7674488349387616 ) ) ;
#43637=CARTESIAN_POINT ( 'NONE',  ( -109.0584444128670185, -294.2617360925467551, -292.9150670596690702 ) ) ;
#43638=CARTESIAN_POINT ( 'NONE',  ( -40.44446316366844485, -298.6656514654368380, -193.4736156261150199 ) ) ;
#43639=CARTESIAN_POINT ( 'NONE',  ( -65.33838767548951409, -275.6864015268652679, -200.7686337656099624 ) ) ;
#43640=CARTESIAN_POINT ( 'NONE',  ( -96.74246357129482021, -290.8962459674995671, -313.1975248219093260 ) ) ;
#43642=CARTESIAN_POINT ( 'NONE',  ( -53.14982046604436761, -295.5936127400568125, -341.7026030798606371 ) ) ;
#43644=CARTESIAN_POINT ( 'NONE',  ( -112.4376424708388100, -280.4445564808393101, -277.2072799755403594 ) ) ;
#43645=CARTESIAN_POINT ( 'NONE',  ( -40.96815612640321547, -278.6922769042372465, -193.9271518185306888 ) ) ;
#43646=CARTESIAN_POINT ( 'NONE',  ( -74.23438386492938434, -282.8775414476518790, -337.8908435394645835 ) ) ;
#43647=CARTESIAN_POINT ( 'NONE',  ( 19.79589733069168744, -275.6004455508007709, -321.8454475181493990 ) ) ;
#43648=CARTESIAN_POINT ( 'NONE',  ( -65.89012771356068754, -281.5083974963083620, -339.1230886815364443 ) ) ;
#43649=CARTESIAN_POINT ( 'NONE',  ( -90.48547601151642539, -277.7149511082502613, -215.6782426686201291 ) ) ;
#43650=CARTESIAN_POINT ( 'NONE',  ( 17.83219048080842484, -278.8397325095853034, -219.3133930364245998 ) ) ;
#43651=CARTESIAN_POINT ( 'NONE',  ( -110.4692925581305190, -271.2345696613039081, -262.1312855415619083 ) ) ;
#43652=CARTESIAN_POINT ( 'NONE',  ( 37.67935169415434871, -277.5796564973703084, -272.4903740196975264 ) ) ;
#43655=CARTESIAN_POINT ( 'NONE',  ( 36.16263112649134825, -291.3594750460984528, -253.7043780236438693 ) ) ;
#43656=CARTESIAN_POINT ( 'NONE',  ( -60.02727588881297294, -289.3382643250567412, -343.9434844327096812 ) ) ;
#43657=CARTESIAN_POINT ( 'NONE',  ( 20.42517514356521247, -276.8896176595218321, -222.2672872807908675 ) ) ;
#43658=CARTESIAN_POINT ( 'NONE',  ( -112.1826874425679534, -270.6241775051232707, -264.7388320909179811 ) ) ;
#43659=CARTESIAN_POINT ( 'NONE',  ( -113.6580699775909693, -283.8613967212689317, -261.4184945825661543 ) ) ;
#43661=CARTESIAN_POINT ( 'NONE',  ( -14.19407528283623954, -284.3520576625339800, -198.9689922327230533 ) ) ;
#43663=CARTESIAN_POINT ( 'NONE',  ( 34.34090954822816855, -292.1393868670133429, -254.5316463890218017 ) ) ;
#43664=CARTESIAN_POINT ( 'NONE',  ( -110.4045761650569233, -282.8631250384627265, -257.1488925995913633 ) ) ;
#43667=CARTESIAN_POINT ( 'NONE',  ( -31.98982391747703957, -290.1194948912177551, -195.5393417737136872 ) ) ;
#43668=CARTESIAN_POINT ( 'NONE',  ( -52.79628683705556114, -281.7264674402689479, -345.1403757092297155 ) ) ;
#43669=CARTESIAN_POINT ( 'NONE',  ( -79.06771080223433046, -279.2250859809200279, -331.2951700798008687 ) ) ;
#43670=CARTESIAN_POINT ( 'NONE',  ( -107.8555923669468513, -285.3727384739846116, -300.4266659618969015 ) ) ;
#43671=CARTESIAN_POINT ( 'NONE',  ( -19.81585606849540682, -286.2838178161671863, -199.4961422187944606 ) ) ;
#43672=CARTESIAN_POINT ( 'NONE',  ( -109.6186008093691981, -279.7955041535999499, -284.2632406269470380 ) ) ;
#43673=CARTESIAN_POINT ( 'NONE',  ( -95.74682072007331612, -279.9727837907842627, -226.2785036770897591 ) ) ;
#43674=CARTESIAN_POINT ( 'NONE',  ( -108.0990636987140192, -286.8743724093508263, -245.4935457620753709 ) ) ;
#43676=CARTESIAN_POINT ( 'NONE',  ( -111.9691736048615098, -296.1475384528994255, -289.3811718663810097 ) ) ;
#43677=CARTESIAN_POINT ( 'NONE',  ( 2.203871065978271204, -290.4995507143703435, -333.6698425052862831 ) ) ;
#43679=CARTESIAN_POINT ( 'NONE',  ( 40.65961533371913106, -278.2662352645559167, -288.1317622949166548 ) ) ;
#43681=CARTESIAN_POINT ( 'NONE',  ( 18.92504472999706522, -292.6587221314950966, -321.8236852042995224 ) ) ;
#43682=CARTESIAN_POINT ( 'NONE',  ( 16.46761851056848869, -288.3544968016658459, -219.9910868476462156 ) ) ;
#43683=CARTESIAN_POINT ( 'NONE',  ( -110.1327145725718850, -280.4865871400288029, -256.9655130582736433 ) ) ;
#43684=CARTESIAN_POINT ( 'NONE',  ( 39.01646439208190742, -289.0279936721215108, -274.3737557109511727 ) ) ;
#43685=CARTESIAN_POINT ( 'NONE',  ( 14.28337524769959543, -289.6601126252392646, -326.8966267918951871 ) ) ;
#43686=CARTESIAN_POINT ( 'NONE',  ( -110.6244322515243397, -286.7579729804272120, -254.3435671289555557 ) ) ;
#43687=CARTESIAN_POINT ( 'NONE',  ( -114.3848676737361814, -278.7032064466724819, -271.6105149549125031 ) ) ;
#43688=CARTESIAN_POINT ( 'NONE',  ( -11.57174894206314519, -292.7991117062976514, -341.4463610709558452 ) ) ;
#43689=CARTESIAN_POINT ( 'NONE',  ( 37.86506954685553694, -281.5928518065873618, -286.9429516643293141 ) ) ;
#43690=CARTESIAN_POINT ( 'NONE',  ( -72.51352105934813608, -275.4422111857547293, -204.9294611848308136 ) ) ;
#43692=CARTESIAN_POINT ( 'NONE',  ( 31.98288692825981272, -290.4805209788416391, -303.7098442033569654 ) ) ;
#43693=CARTESIAN_POINT ( 'NONE',  ( -80.65414666818847422, -271.7138339291482794, -207.8633558666442411 ) ) ;
#43695=CARTESIAN_POINT ( 'NONE',  ( -108.3479958752068910, -278.2866447170324022, -253.1537240446308203 ) ) ;
#43696=CARTESIAN_POINT ( 'NONE',  ( 27.32192974589782253, -277.2993627368304601, -311.5282727642073155 ) ) ;
#43697=CARTESIAN_POINT ( 'NONE',  ( -68.31191880699030605, -299.0624760743460229, -203.5924135421674350 ) ) ;
#43698=CARTESIAN_POINT ( 'NONE',  ( -52.88173496771922544, -282.3052442659360963, -345.5907572744412164 ) ) ;
#43699=CARTESIAN_POINT ( 'NONE',  ( -109.3308917424071325, -292.0886000120624999, -287.5521129261514375 ) ) ;
#43700=CARTESIAN_POINT ( 'NONE',  ( -104.6512379963110959, -298.5422759200166638, -234.3027117457391455 ) ) ;
#43701=CARTESIAN_POINT ( 'NONE',  ( -34.08346385356971808, -299.2971614199084343, -193.7575374131689898 ) ) ;
#43702=CARTESIAN_POINT ( 'NONE',  ( -9.791947028515874507, -296.6916292587238786, -339.9386972112981766 ) ) ;
#43703=CARTESIAN_POINT ( 'NONE',  ( -34.80939034443976965, -281.0201362934014355, -345.1643467824383720 ) ) ;
#43704=CARTESIAN_POINT ( 'NONE',  ( -81.91468632816209094, -291.1295882377192470, -207.5997190764420850 ) ) ;
#43705=CARTESIAN_POINT ( 'NONE',  ( -4.563534688456956978, -272.5062558468840166, -203.2840338853002038 ) ) ;
#43706=CARTESIAN_POINT ( 'NONE',  ( -37.99623278272093074, -287.6442016318833339, -194.1639263970458273 ) ) ;
#43707=CARTESIAN_POINT ( 'NONE',  ( -98.37561611982357590, -288.9108841644597305, -310.9929316632356517 ) ) ;
#43708=CARTESIAN_POINT ( 'NONE',  ( -93.98250134251853183, -240.8842209496550595, -341.6624768569019466 ) ) ;
#43710=CARTESIAN_POINT ( 'NONE',  ( -95.95087428743453017, -288.4618411036333328, -319.4076465295094636 ) ) ;
#43711=CARTESIAN_POINT ( 'NONE',  ( -26.47593335298036266, -288.5769298078166116, -342.6203711738583593 ) ) ;
#43713=CARTESIAN_POINT ( 'NONE',  ( -29.50823570249005456, -287.2288385172611811, -194.0713457680148792 ) ) ;
#43714=CARTESIAN_POINT ( 'NONE',  ( -83.01667858534520406, -278.0302404586508942, -327.3988506369762490 ) ) ;
#43715=CARTESIAN_POINT ( 'NONE',  ( 39.13385699784925720, -292.4003695617886365, -264.6181508617400482 ) ) ;
#43716=CARTESIAN_POINT ( 'NONE',  ( -93.35159915019727350, -284.4832558853427145, -323.0701152733925596 ) ) ;
#43717=CARTESIAN_POINT ( 'NONE',  ( 29.16717837900045751, -283.5632175286992833, -307.8757635461401492 ) ) ;
#43718=CARTESIAN_POINT ( 'NONE',  ( -37.30999888295170308, -283.3850083620802138, -347.3530293155156983 ) ) ;
#43720=CARTESIAN_POINT ( 'NONE',  ( -9.243131624974672889, -280.7632035454689117, -202.9626169985295689 ) ) ;
#43721=CARTESIAN_POINT ( 'NONE',  ( -83.97320365025282740, -219.6140998129361321, -352.5802664969301645 ) ) ;
#43722=CARTESIAN_POINT ( 'NONE',  ( -90.97752918039822134, -229.6550970709923263, -347.1063063428075566 ) ) ;
#43723=CARTESIAN_POINT ( 'NONE',  ( 24.24861201465908422, -23.26907645984904605, -341.8364469676749877 ) ) ;
#43724=CARTESIAN_POINT ( 'NONE',  ( -97.97128717005418252, -272.3182944487887767, -229.3237794709698392 ) ) ;
#43725=CARTESIAN_POINT ( 'NONE',  ( -37.69499331564374245, -294.5640847617744953, -347.3118364924222874 ) ) ;
#43726=CARTESIAN_POINT ( 'NONE',  ( 194.0023159067837923, 275.6218090567761010, -124.1595538786234272 ) ) ;
#43727=CARTESIAN_POINT ( 'NONE',  ( -93.77014500029007138, -271.9444184519718419, -218.6781672612716818 ) ) ;
#43728=CARTESIAN_POINT ( 'NONE',  ( -108.6523958401421197, -298.6809050814571265, -249.7298272196343873 ) ) ;
#43729=CARTESIAN_POINT ( 'NONE',  ( 24.66333943354051783, -289.4091649891917086, -309.8151234404397769 ) ) ;
#43731=CARTESIAN_POINT ( 'NONE',  ( -30.59964104961693820, -295.9101165365055977, -346.8291822462352343 ) ) ;
#43732=CARTESIAN_POINT ( 'NONE',  ( -39.98241614098324703, -286.5104276740514138, -197.3473175010811076 ) ) ;
#43733=CARTESIAN_POINT ( 'NONE',  ( -85.60300669407659768, -272.3224516986533104, -210.7596180231304857 ) ) ;
#43734=CARTESIAN_POINT ( 'NONE',  ( -16.54074434826786089, -295.5929805137505468, -344.3856840888263946 ) ) ;
#43735=CARTESIAN_POINT ( 'NONE',  ( 34.39637747893767994, -294.3970498302081182, -298.1671447456228634 ) ) ;
#43736=CARTESIAN_POINT ( 'NONE',  ( -65.32892295345830291, -291.8425571907436620, -202.9256831570402539 ) ) ;
#43738=CARTESIAN_POINT ( 'NONE',  ( -21.67762877955538414, -276.1715921763665165, -196.4425745448380383 ) ) ;
#43739=CARTESIAN_POINT ( 'NONE',  ( 37.78991065937461968, -274.5349149004036349, -285.3026634259592242 ) ) ;
#43741=CARTESIAN_POINT ( 'NONE',  ( -111.2763734306744823, -278.3269299897797850, -249.0728351266827190 ) ) ;
#43742=CARTESIAN_POINT ( 'NONE',  ( 36.17707836545140054, -273.8607265000895268, -263.3649551639949777 ) ) ;
#43743=CARTESIAN_POINT ( 'NONE',  ( -48.93783186929407947, -274.9807740408643895, -197.9235692558317794 ) ) ;
#43744=CARTESIAN_POINT ( 'NONE',  ( 17.45365612282845547, -275.8006207662948555, -221.6971292762044925 ) ) ;
#43745=CARTESIAN_POINT ( 'NONE',  ( -37.62534918568967868, -299.6487773713902811, -194.1616431679639447 ) ) ;
#43746=CARTESIAN_POINT ( 'NONE',  ( -9.836181847668704847, -274.7147857051502342, -340.5170390964740363 ) ) ;
#43747=CARTESIAN_POINT ( 'NONE',  ( -41.03608490611206605, -295.7512518029748207, -343.3822242119767907 ) ) ;
#43748=CARTESIAN_POINT ( 'NONE',  ( -15.43458616841937925, -293.3378237969102429, -340.6674952301746657 ) ) ;
#43750=CARTESIAN_POINT ( 'NONE',  ( -93.28493400725571405, -278.3220086836903420, -323.2568890638909238 ) ) ;
#43752=CARTESIAN_POINT ( 'NONE',  ( 22.27960606024607415, -275.1306188513710254, -228.2170412931611736 ) ) ;
#43753=CARTESIAN_POINT ( 'NONE',  ( -102.0921358743618867, -283.7740724592304105, -229.6096843534307084 ) ) ;
#43754=CARTESIAN_POINT ( 'NONE',  ( -111.3931695871596474, -298.3832841303209307, -283.5546141073987769 ) ) ;
#43756=CARTESIAN_POINT ( 'NONE',  ( -96.69986180757408079, -284.3463487260885358, -227.5704808760709739 ) ) ;
#43757=CARTESIAN_POINT ( 'NONE',  ( -108.1907348321117865, -277.0715952243014044, -248.9511134139237072 ) ) ;
#43758=CARTESIAN_POINT ( 'NONE',  ( -87.51038438886374138, -276.3437488854533512, -324.1986331141633855 ) ) ;
#43759=CARTESIAN_POINT ( 'NONE',  ( 15.73214179078694031, -284.3014756628151645, -323.4251477768797827 ) ) ;
#43761=CARTESIAN_POINT ( 'NONE',  ( 35.99953040875986687, -276.8091609505043493, -274.3188249778099816 ) ) ;
#43763=CARTESIAN_POINT ( 'NONE',  ( 38.34051367161838186, -274.0696763626419283, -279.6705962231586113 ) ) ;
#43764=CARTESIAN_POINT ( 'NONE',  ( -70.45057094878701776, -281.6168532638089346, -202.8790381081299472 ) ) ;
#43766=CARTESIAN_POINT ( 'NONE',  ( 11.50391496486480136, -290.3008337343053427, -328.0102296968251494 ) ) ;
#43767=CARTESIAN_POINT ( 'NONE',  ( -35.84621781830518472, -290.0707210140669758, -195.3633988938459254 ) ) ;
#43769=CARTESIAN_POINT ( 'NONE',  ( -50.00743799356180119, -296.6818433214320976, -198.0651320073855572 ) ) ;
#43770=CARTESIAN_POINT ( 'NONE',  ( -88.76950513434790935, -289.4608596972686883, -216.7546326809274149 ) ) ;
#43771=CARTESIAN_POINT ( 'NONE',  ( -114.4693872376281121, -273.8646567567205921, -270.3778293100139649 ) ) ;
#43773=CARTESIAN_POINT ( 'NONE',  ( -17.91964510196394045, -287.2860126728338059, -344.1546917510391950 ) ) ;
#43774=CARTESIAN_POINT ( 'NONE',  ( -40.74830541753437529, -284.2498549853416989, -194.3993411138964689 ) ) ;
#43775=CARTESIAN_POINT ( 'NONE',  ( -15.94397345712669711, -284.1951816980555918, -340.7707210863141540 ) ) ;
#43776=CARTESIAN_POINT ( 'NONE',  ( -82.88727644386374038, -284.4961380497286996, -327.6817052116827540 ) ) ;
#43777=CARTESIAN_POINT ( 'NONE',  ( -100.9000991719601785, -291.9886904965841268, -310.9384064725188068 ) ) ;
#43778=CIRCLE ( 'NONE', #51349, 6.154241149514405151 ) ;
#43779=CARTESIAN_POINT ( 'NONE',  ( -24.16740299958334504, -274.5491193215861472, -194.4638250408869453 ) ) ;
#43780=CARTESIAN_POINT ( 'NONE',  ( -100.4672205133025500, -289.1894175438212073, -228.7403770448274543 ) ) ;
#43781=CARTESIAN_POINT ( 'NONE',  ( -104.9755861778273527, -278.0758623858064311, -307.1667895266301116 ) ) ;
#43783=CARTESIAN_POINT ( 'NONE',  ( 7.061155533618573621, -296.4244801106389673, -330.4274920493517698 ) ) ;
#43785=CARTESIAN_POINT ( 'NONE',  ( -69.85430415644619018, -291.9805209788416391, -337.9475929042657754 ) ) ;
#43786=CARTESIAN_POINT ( 'NONE',  ( -68.00529112903117834, -282.1482339243575552, -337.1517435699443013 ) ) ;
#43787=CARTESIAN_POINT ( 'NONE',  ( -103.3774047792883835, -276.0760238957922184, -306.2681386755523363 ) ) ;
#43788=CARTESIAN_POINT ( 'NONE',  ( -69.81892380619837013, -272.1121676740978614, -201.2965808681847193 ) ) ;
#43789=CARTESIAN_POINT ( 'NONE',  ( 35.70334259924545961, -274.9529708153341971, -274.3264179702936758 ) ) ;
#43790=CARTESIAN_POINT ( 'NONE',  ( -3.333343410057451717, -294.0299275527530654, -204.9842151243176147 ) ) ;
#43791=CARTESIAN_POINT ( 'NONE',  ( 35.87769660338809530, -294.5345142554991185, -273.4870979987965143 ) ) ;
#43792=CARTESIAN_POINT ( 'NONE',  ( -34.99681943398362449, -293.5062945300277875, -193.9732830840702036 ) ) ;
#43793=CARTESIAN_POINT ( 'NONE',  ( 39.11467311429223059, -294.9023003633832900, -273.1398338931202261 ) ) ;
#43794=CARTESIAN_POINT ( 'NONE',  ( -110.2417807778729610, -296.3351033581044476, -274.1792648812389075 ) ) ;
#43795=CARTESIAN_POINT ( 'NONE',  ( -73.29585713263305990, -291.5291735445060795, -336.1813219064975442 ) ) ;
#43796=CARTESIAN_POINT ( 'NONE',  ( -86.10073152399561991, -283.8737515159365898, -329.9560578836664604 ) ) ;
#43797=CARTESIAN_POINT ( 'NONE',  ( -92.26023765429999912, -271.4169159960144952, -218.1477504421173705 ) ) ;
#43798=CARTESIAN_POINT ( 'NONE',  ( -29.46082735709656220, -285.9826880334969701, -193.7654794065425392 ) ) ;
#43799=CARTESIAN_POINT ( 'NONE',  ( -97.40175962688509514, -279.9242146781659244, -314.7067488803897390 ) ) ;
#43800=CARTESIAN_POINT ( 'NONE',  ( -94.42120560891630987, -283.9963229609776931, -224.1994599312868388 ) ) ;
#43801=CARTESIAN_POINT ( 'NONE',  ( -9.012805263682816204, -286.6815371362696396, -339.8190490488023556 ) ) ;
#43802=CARTESIAN_POINT ( 'NONE',  ( -66.85903145171967310, -277.8090417662626805, -200.5826640474423073 ) ) ;
#43803=CARTESIAN_POINT ( 'NONE',  ( -71.74250447947856912, -195.9422791308210492, -360.7315132586310824 ) ) ;
#43804=CARTESIAN_POINT ( 'NONE',  ( -73.58071125799985168, -285.0649747014736590, -206.9059095468134899 ) ) ;
#43805=CARTESIAN_POINT ( 'NONE',  ( 37.75931178895508111, -282.9469798533269795, -285.4557106854428525 ) ) ;
#43806=CARTESIAN_POINT ( 'NONE',  ( -12.31181026184407656, -287.7932266541396871, -342.9862634846128344 ) ) ;
#43807=CARTESIAN_POINT ( 'NONE',  ( -56.70090291831119345, -278.8976790862839721, -344.1154021804333638 ) ) ;
#43808=CARTESIAN_POINT ( 'NONE',  ( -41.34180558713192255, -278.4166650084789012, -346.7764505700321251 ) ) ;
#43809=CARTESIAN_POINT ( 'NONE',  ( -67.30434741400488008, -279.4812824095527048, -203.7799539836873635 ) ) ;
#43810=CARTESIAN_POINT ( 'NONE',  ( -54.61611036000540764, -275.8089637426986656, -197.7426523508493119 ) ) ;
#43811=CARTESIAN_POINT ( 'NONE',  ( 37.09656688678564507, -293.7987332985782700, -290.0574223014764357 ) ) ;
#43812=CARTESIAN_POINT ( 'NONE',  ( 30.91920072636273176, -285.9712982299749910, -300.6935030813089611 ) ) ;
#43813=CARTESIAN_POINT ( 'NONE',  ( -98.57402308712372019, -292.7617565300981255, -224.9846160179839387 ) ) ;
#43814=CARTESIAN_POINT ( 'NONE',  ( -103.9939258800449551, -295.8838608825694223, -239.7151103725387031 ) ) ;
#43815=CARTESIAN_POINT ( 'NONE',  ( 34.92927226068994173, -293.0811880218096235, -259.9210970647380918 ) ) ;
#43817=CARTESIAN_POINT ( 'NONE',  ( -44.88039979122734024, -293.0386417588241557, -193.9889443561916380 ) ) ;
#43818=CARTESIAN_POINT ( 'NONE',  ( 33.75122589752545821, -282.4284805786579113, -287.4346365581382088 ) ) ;
#43819=CARTESIAN_POINT ( 'NONE',  ( -20.58003824011520777, -297.1777206810681946, -193.6732168222712289 ) ) ;
#43820=CARTESIAN_POINT ( 'NONE',  ( -97.20548749604594718, -290.5554468493023137, -318.6482230603169228 ) ) ;
#43821=CARTESIAN_POINT ( 'NONE',  ( -109.5162230189088604, -282.3967838770487333, -293.4505001835232179 ) ) ;
#43822=CARTESIAN_POINT ( 'NONE',  ( 14.59257516847157277, -288.6783778740298203, -327.2539087294928777 ) ) ;
#43823=CARTESIAN_POINT ( 'NONE',  ( -67.56032080925972139, -285.9776975331199651, -203.8861418563127472 ) ) ;
#43825=CARTESIAN_POINT ( 'NONE',  ( -32.49377328605026349, -123.7660681094353947, -362.0747317338332891 ) ) ;
#43826=CARTESIAN_POINT ( 'NONE',  ( 138.3761275019903678, 178.4032963545091661, -238.2084800396306434 ) ) ;
#43827=CARTESIAN_POINT ( 'NONE',  ( -99.59977877579785854, -278.2791676133982719, -231.8388061061633323 ) ) ;
#43828=CARTESIAN_POINT ( 'NONE',  ( -7.862580350387181838, -279.3680559078222245, -203.2265432578485331 ) ) ;
#43829=CARTESIAN_POINT ( 'NONE',  ( 33.69567661556746430, -274.8400821527634434, -240.5681502228325712 ) ) ;
#43830=CARTESIAN_POINT ( 'NONE',  ( -101.2059816391420384, -255.8329364732449562, -325.0564836861664730 ) ) ;
#43831=CARTESIAN_POINT ( 'NONE',  ( -102.8966756669376394, -277.6439150704397889, -231.0007761553897296 ) ) ;
#43832=CARTESIAN_POINT ( 'NONE',  ( -34.81557612609163499, -281.0404013122154652, -344.9758826556931695 ) ) ;
#43833=CARTESIAN_POINT ( 'NONE',  ( 24.89770203432625095, -295.8966208393606507, -313.9754723689898697 ) ) ;
#43834=CARTESIAN_POINT ( 'NONE',  ( -64.09998110935865157, -292.1858064316247123, -202.3624066501358811 ) ) ;
#43835=CARTESIAN_POINT ( 'NONE',  ( -53.53336389100431347, -287.9490785076002339, -342.0484495073671951 ) ) ;
#43836=CARTESIAN_POINT ( 'NONE',  ( 34.62343721330418589, -275.8602680037275263, -243.2625609396641266 ) ) ;
#43837=CARTESIAN_POINT ( 'NONE',  ( -94.77212354698522745, -296.0833769705415648, -315.4249224209679028 ) ) ;
#43841=CARTESIAN_POINT ( 'NONE',  ( -56.22094678245019850, -281.7310865348313769, -197.1437061014673020 ) ) ;
#43844=CARTESIAN_POINT ( 'NONE',  ( 31.35517082314290960, -282.2901848812873595, -244.6232522593568035 ) ) ;
#43845=CARTESIAN_POINT ( 'NONE',  ( -113.0366189709563685, -280.4038966261870769, -263.1329113806338000 ) ) ;
#43846=CIRCLE ( 'NONE', #15147, 2.395975569037644970 ) ;
#43847=CARTESIAN_POINT ( 'NONE',  ( 35.93810580643082631, -280.6236185276035258, -271.3287905638847519 ) ) ;
#43848=CARTESIAN_POINT ( 'NONE',  ( -96.82970168000497324, -271.6364068563615888, -226.7805554554041976 ) ) ;
#43851=CARTESIAN_POINT ( 'NONE',  ( 35.57347531852190770, -276.0473129241058814, -245.9543226703549976 ) ) ;
#43852=ORIENTED_EDGE ( 'NONE', *, *, #36263, .T. ) ;
#43853=CARTESIAN_POINT ( 'NONE',  ( 35.34057441301066405, -277.3146272655753819, -251.8601012629020488 ) ) ;
#43854=CARTESIAN_POINT ( 'NONE',  ( -110.1111417280659595, -276.8296458870128163, -293.8385715257469997 ) ) ;
#43857=CARTESIAN_POINT ( 'NONE',  ( -106.7030853027152517, -286.1474302321784080, -299.9462420806698901 ) ) ;
#43858=CARTESIAN_POINT ( 'NONE',  ( -86.02888094471506975, -290.5541441838533956, -215.6837797720032484 ) ) ;
#43860=CARTESIAN_POINT ( 'NONE',  ( 25.46664965313900808, -286.3126007077700024, -225.9714876793367182 ) ) ;
#43861=CARTESIAN_POINT ( 'NONE',  ( -29.35730981752316282, -281.1896220680601459, -343.9937296700563820 ) ) ;
#43862=CARTESIAN_POINT ( 'NONE',  ( -89.32325833297035445, -282.3759773022986792, -322.5219354054040082 ) ) ;
#43863=CARTESIAN_POINT ( 'NONE',  ( 26.19223815266872890, -285.1079081965983164, -231.5699735935411638 ) ) ;
#43864=CARTESIAN_POINT ( 'NONE',  ( -18.61961892768315607, -284.0108196002487375, -341.3829175781882554 ) ) ;
#43865=CARTESIAN_POINT ( 'NONE',  ( 24.51000108298645941, -272.9770163698478314, -227.9193896109121056 ) ) ;
#43866=CARTESIAN_POINT ( 'NONE',  ( -89.32543927409190587, -283.7351082154200981, -214.5746402815611020 ) ) ;
#43867=CARTESIAN_POINT ( 'NONE',  ( -87.25491953841047632, -297.7475330837379488, -326.4099424918628074 ) ) ;
#43868=CARTESIAN_POINT ( 'NONE',  ( -67.41383070060905425, -280.5890352419417013, -203.5711578420643093 ) ) ;
#43869=CARTESIAN_POINT ( 'NONE',  ( -77.56347038069934285, -287.5138048358635956, -206.8612154386999862 ) ) ;
#43872=CARTESIAN_POINT ( 'NONE',  ( 38.00329673141931153, -295.3997119000199518, -264.6650101750379349 ) ) ;
#43873=CARTESIAN_POINT ( 'NONE',  ( -102.3282010876691857, -276.0511314031393226, -307.9055066036429480 ) ) ;
#43874=CARTESIAN_POINT ( 'NONE',  ( -43.18024462896039495, -288.3212798056808879, -346.9775014694620836 ) ) ;
#43875=CARTESIAN_POINT ( 'NONE',  ( 36.42157156636137927, -291.9216372805134370, -268.0329938335682982 ) ) ;
#43876=CARTESIAN_POINT ( 'NONE',  ( -109.3672217190964489, -277.4292911423320902, -255.6840360473692328 ) ) ;
#43877=CARTESIAN_POINT ( 'NONE',  ( -110.5854241665983011, -294.5348705711824664, -282.4533622045860284 ) ) ;
#43878=EDGE_CURVE ( 'NONE', #71834, #42078, #72332, .T. ) ;
#43879=CARTESIAN_POINT ( 'NONE',  ( -44.36388845285280524, -293.2767947673993376, -197.1530539317977002 ) ) ;
#43880=CARTESIAN_POINT ( 'NONE',  ( -110.4542110544635705, -280.8376638359844719, -287.0812184334320705 ) ) ;
#43881=CARTESIAN_POINT ( 'NONE',  ( 14.98901086110268466, -292.8098213345518843, -325.8967321303628637 ) ) ;
#43882=CARTESIAN_POINT ( 'NONE',  ( 30.69143273250614001, -288.7711097746224596, -241.6293308995907694 ) ) ;
#43883=CARTESIAN_POINT ( 'NONE',  ( -112.3632089389286932, -288.6390166940348081, -282.4336997310314814 ) ) ;
#43884=CARTESIAN_POINT ( 'NONE',  ( -56.19921102510999589, -290.7250158839274832, -341.5461504259332628 ) ) ;
#43886=CARTESIAN_POINT ( 'NONE',  ( -109.0950958847691084, -291.1661216797250518, -284.7098272671286168 ) ) ;
#43888=CARTESIAN_POINT ( 'NONE',  ( 14.34715685954928155, -289.5500320692665355, -326.9685827087948269 ) ) ;
#43889=CARTESIAN_POINT ( 'NONE',  ( -91.86584065268043275, -277.2996716465107738, -218.2719317715601903 ) ) ;
#43890=CARTESIAN_POINT ( 'NONE',  ( -25.40305715213583326, -280.5336310240380726, -194.3136782140570915 ) ) ;
#43891=CARTESIAN_POINT ( 'NONE',  ( 25.08765291017316912, -281.8164502604197423, -315.4203676390355326 ) ) ;
#43892=CARTESIAN_POINT ( 'NONE',  ( 37.26648167704814796, -285.4536822679012289, -262.7047575499842651 ) ) ;
#43893=CARTESIAN_POINT ( 'NONE',  ( 121.3395553409046528, -299.5541904835127980, -191.8695490883551713 ) ) ;
#43894=CARTESIAN_POINT ( 'NONE',  ( 35.27840652580110969, -279.4911956604726129, -254.8996255427316555 ) ) ;
#43895=CARTESIAN_POINT ( 'NONE',  ( -8.823591980929922585, -280.6790647675518358, -339.7827283724313929 ) ) ;
#43896=CARTESIAN_POINT ( 'NONE',  ( 6.586621361128567109, -59.71314100781844303, -351.1713062918258856 ) ) ;
#43897=CARTESIAN_POINT ( 'NONE',  ( -112.6183987848659882, -276.8743466793583821, -282.8561727090163913 ) ) ;
#43898=CARTESIAN_POINT ( 'NONE',  ( -109.6811053818439063, -283.7950369421499204, -244.8953967701154966 ) ) ;
#43899=CARTESIAN_POINT ( 'NONE',  ( -33.80982893058406091, -299.0386861120962863, -197.1252400388727324 ) ) ;
#43900=CARTESIAN_POINT ( 'NONE',  ( -90.40554557003881087, -292.8853601168768250, -219.0710729265712473 ) ) ;
#43901=CARTESIAN_POINT ( 'NONE',  ( -34.79678551239572926, -299.3985538800711197, -193.8537097873024209 ) ) ;
#43902=CARTESIAN_POINT ( 'NONE',  ( 35.66413123561213183, -275.1991483550519320, -268.8657673294840151 ) ) ;
#43903=CARTESIAN_POINT ( 'NONE',  ( -41.11504517770968192, -297.0997812010708117, -345.2790530161220204 ) ) ;
#43904=CARTESIAN_POINT ( 'NONE',  ( -20.49433778279724194, -289.0083751281943591, -345.5501079595523493 ) ) ;
#43905=CARTESIAN_POINT ( 'NONE',  ( 27.06453089242522125, -280.1592517947494230, -309.9716337614506187 ) ) ;
#43906=CARTESIAN_POINT ( 'NONE',  ( -34.95828677764342984, -291.9145995763387305, -193.3848641482099140 ) ) ;
#43908=CARTESIAN_POINT ( 'NONE',  ( -110.3582582412613959, -289.5283560155095870, -276.6381833524913532 ) ) ;
#43909=CARTESIAN_POINT ( 'NONE',  ( -9.163716676360019520, -292.6837187567485898, -339.9215321763049928 ) ) ;
#43912=CARTESIAN_POINT ( 'NONE',  ( -105.1725115110989748, -289.6951503130741230, -297.6441111635741663 ) ) ;
#43915=CARTESIAN_POINT ( 'NONE',  ( -65.80130370130943618, -286.6301033374155054, -199.0527479502372330 ) ) ;
#43916=CARTESIAN_POINT ( 'NONE',  ( -37.30987171927208124, -297.5519495502701375, -340.3611179825599606 ) ) ;
#43917=CARTESIAN_POINT ( 'NONE',  ( -58.79708573511451419, -294.3816905464427123, -344.1219272551581980 ) ) ;
#43918=CARTESIAN_POINT ( 'NONE',  ( -55.56836374640140974, -284.5971615363647516, -344.6651354027273442 ) ) ;
#43919=CARTESIAN_POINT ( 'NONE',  ( -99.60820917864782587, -284.9116670769285520, -232.1612445117027335 ) ) ;
#43920=CARTESIAN_POINT ( 'NONE',  ( 30.74115971296555827, -277.2371678003347597, -298.1727273250932058 ) ) ;
#43921=CARTESIAN_POINT ( 'NONE',  ( -31.49819311935199551, -292.9982499648074281, -344.8280862273466596 ) ) ;
#43922=CARTESIAN_POINT ( 'NONE',  ( 3.341517111109728155, -275.2866304013976446, -331.4512672638328468 ) ) ;
#43925=CARTESIAN_POINT ( 'NONE',  ( -13.79254825091533476, -294.4213891932420779, -343.6494645141034994 ) ) ;
#43926=CARTESIAN_POINT ( 'NONE',  ( 33.63945168365759741, -289.1802533405262920, -247.8910439658979783 ) ) ;
#43927=CARTESIAN_POINT ( 'NONE',  ( -112.3013091418980167, -297.8360021364579211, -254.0963911939644220 ) ) ;
#43928=CARTESIAN_POINT ( 'NONE',  ( 35.37494195359314375, -288.1048286698856487, -262.8656105004017149 ) ) ;
#43929=CARTESIAN_POINT ( 'NONE',  ( -114.1421496237037303, -277.6313979254216520, -268.7272552213032100 ) ) ;
#43930=CARTESIAN_POINT ( 'NONE',  ( -37.68019307119700301, -295.7076600064600598, -347.2715017254911913 ) ) ;
#43931=CARTESIAN_POINT ( 'NONE',  ( 2.509953869632158163, -286.6639971934728237, -334.8598390977539907 ) ) ;
#43932=CARTESIAN_POINT ( 'NONE',  ( -103.0953205865691444, -296.3626100400822452, -310.3886795879174088 ) ) ;
#43933=CARTESIAN_POINT ( 'NONE',  ( -107.0230643449753813, -291.1751839049461523, -248.4879330637774899 ) ) ;
#43935=CARTESIAN_POINT ( 'NONE',  ( -110.6395504398199847, -271.5021483123970825, -270.3477634379551660 ) ) ;
#43936=CARTESIAN_POINT ( 'NONE',  ( 45.91229879761790045, 10.79500447389408180, -328.5722265924176781 ) ) ;
#43937=CARTESIAN_POINT ( 'NONE',  ( 38.09716837992449001, -288.9263545765463164, -258.7988615211872911 ) ) ;
#43938=CARTESIAN_POINT ( 'NONE',  ( -99.86837403722181250, -282.6952119285918457, -220.4570493818173702 ) ) ;
#43939=ORIENTED_EDGE ( 'NONE', *, *, #49884, .T. ) ;
#43940=CARTESIAN_POINT ( 'NONE',  ( -36.74500289911770778, -279.4080578690017092, -193.4523371623326113 ) ) ;
#43941=CARTESIAN_POINT ( 'NONE',  ( -86.03591476719596187, -285.7291711703344390, -327.1845452309248117 ) ) ;
#43942=CARTESIAN_POINT ( 'NONE',  ( -103.5209802914841504, -283.6284706816451262, -232.0602697252504925 ) ) ;
#43943=CARTESIAN_POINT ( 'NONE',  ( 18.89769419500824199, -286.3143098734357750, -319.2075638371107402 ) ) ;
#43944=CARTESIAN_POINT ( 'NONE',  ( 24.30780988661840425, -276.8193802305753479, -226.2975501514406744 ) ) ;
#43945=CARTESIAN_POINT ( 'NONE',  ( -98.50251896629556825, -297.5990085793167168, -230.3027847154496897 ) ) ;
#43946=CARTESIAN_POINT ( 'NONE',  ( 16.50916399327210371, -292.9510359774853896, -320.3743953365233210 ) ) ;
#43947=CARTESIAN_POINT ( 'NONE',  ( -69.92674118574088027, -280.2856268490990033, -200.6938370308662343 ) ) ;
#43948=CARTESIAN_POINT ( 'NONE',  ( -32.42055882953000179, -276.9885209775325166, -343.2450212210904965 ) ) ;
#43949=CARTESIAN_POINT ( 'NONE',  ( -100.8963426182330210, -278.3947543979291481, -234.2404855700987127 ) ) ;
#43950=CARTESIAN_POINT ( 'NONE',  ( 13.74826779946631206, -275.8279046361241740, -213.0948172545879800 ) ) ;
#43951=CARTESIAN_POINT ( 'NONE',  ( -91.12211186784148254, -276.7146977730510002, -325.1087081909852259 ) ) ;
#43952=CARTESIAN_POINT ( 'NONE',  ( 184.9426652459076479, 263.7189940584568717, -153.2499980067237004 ) ) ;
#43953=CARTESIAN_POINT ( 'NONE',  ( -90.16780180670041034, -275.7983667034246196, -323.6718310210713412 ) ) ;
#43954=CARTESIAN_POINT ( 'NONE',  ( -107.8244491619790466, -297.5976398315835922, -300.0071060735955939 ) ) ;
#43957=CARTESIAN_POINT ( 'NONE',  ( 139.3989977797154154, 177.7276089766264704, -238.0725708408485843 ) ) ;
#43958=CARTESIAN_POINT ( 'NONE',  ( -70.13298351644149875, -286.6893129412501935, -204.7806756150225453 ) ) ;
#43959=CARTESIAN_POINT ( 'NONE',  ( -98.54161512224210639, -286.9195954354957507, -225.2351453106712995 ) ) ;
#43960=CARTESIAN_POINT ( 'NONE',  ( 27.75268061214526938, -286.4480740683131330, -236.9836725831424928 ) ) ;
#43961=CARTESIAN_POINT ( 'NONE',  ( -109.8329067194844271, -276.7705925798484827, -284.2650860842762199 ) ) ;
#43962=CARTESIAN_POINT ( 'NONE',  ( -110.4130066558641232, -286.5833557021732076, -257.1956025475437855 ) ) ;
#43963=CARTESIAN_POINT ( 'NONE',  ( -39.70424885127346926, -278.5018550133532358, -196.6930236565489736 ) ) ;
#43964=CARTESIAN_POINT ( 'NONE',  ( -94.82837353542690551, -279.2247955445440084, -316.1690498192689915 ) ) ;
#43965=CARTESIAN_POINT ( 'NONE',  ( 23.84160967976788470, -275.4916201576054391, -230.4287871889740700 ) ) ;
#43966=CARTESIAN_POINT ( 'NONE',  ( 38.69447677087688220, -286.4693588440511576, -280.0880675028896007 ) ) ;
#43967=CARTESIAN_POINT ( 'NONE',  ( 20.00135078341185135, -281.6599002731761630, -219.1951413971889622 ) ) ;
#43968=CARTESIAN_POINT ( 'NONE',  ( -31.63459242285705031, -283.4743027276146563, -347.1008754879867979 ) ) ;
#43972=CARTESIAN_POINT ( 'NONE',  ( -56.94803817897030740, -291.1626689396801453, -343.5993280237652243 ) ) ;
#43973=CARTESIAN_POINT ( 'NONE',  ( -71.70010641476484636, -288.1814959839315975, -338.7189865275929606 ) ) ;
#43974=CARTESIAN_POINT ( 'NONE',  ( -94.04252156878439450, -297.4541001079250577, -321.2869098794395768 ) ) ;
#43975=CARTESIAN_POINT ( 'NONE',  ( -39.16211993168021621, -297.2259266605749986, -197.2098559609576398 ) ) ;
#43978=CARTESIAN_POINT ( 'NONE',  ( 22.13569942842645233, -292.2453615147028927, -221.6194342911086608 ) ) ;
#43979=CARTESIAN_POINT ( 'NONE',  ( 24.12294964675093212, -285.4722109202510296, -229.6139952526254433 ) ) ;
#43980=CARTESIAN_POINT ( 'NONE',  ( -49.83805983295521713, -290.1305635207045270, -197.3583107231216616 ) ) ;
#43981=CARTESIAN_POINT ( 'NONE',  ( -3.167891246722748022, -289.7956196537449500, -335.3734094343310517 ) ) ;
#43982=CARTESIAN_POINT ( 'NONE',  ( 21.27581636871892101, -295.4090924074130839, -223.5744983911110353 ) ) ;
#43983=CARTESIAN_POINT ( 'NONE',  ( 28.61627507404245563, -290.0276912192342706, -306.1705853382319447 ) ) ;
#43984=CARTESIAN_POINT ( 'NONE',  ( -3.899829629486747606, -286.6120053630060625, -337.6930739801743471 ) ) ;
#43986=CARTESIAN_POINT ( 'NONE',  ( -29.78056737124442677, -290.9567199945363996, -345.0304473626831623 ) ) ;
#43987=CARTESIAN_POINT ( 'NONE',  ( -109.8468582027819878, -285.6290503384535668, -260.0455714260510831 ) ) ;
#43988=CARTESIAN_POINT ( 'NONE',  ( 35.96747810008972834, -295.3388831340281513, -253.6964863504453263 ) ) ;
#43991=CARTESIAN_POINT ( 'NONE',  ( -54.97374857452631147, -275.8064216708332310, -197.0977733460076138 ) ) ;
#43992=CARTESIAN_POINT ( 'NONE',  ( -13.48635367079022451, -281.9316368217291142, -339.5778642325623764 ) ) ;
#43993=CARTESIAN_POINT ( 'NONE',  ( -71.13837325483054030, -281.4980089448363856, -337.3290889095470675 ) ) ;
#43994=CARTESIAN_POINT ( 'NONE',  ( -110.6488173352366857, -295.4588708060402382, -293.4318003339238885 ) ) ;
#43995=CARTESIAN_POINT ( 'NONE',  ( -108.9142837430079709, -271.0398311269453870, -251.3143658052405840 ) ) ;
#43996=CARTESIAN_POINT ( 'NONE',  ( -46.10135080718824696, -275.2438111847399114, -344.3355590814085190 ) ) ;
#43997=CARTESIAN_POINT ( 'NONE',  ( -98.86954993854234885, -298.4217027132953035, -230.0748759432026702 ) ) ;
#43999=CARTESIAN_POINT ( 'NONE',  ( -50.31683694748694080, -293.4553212652793377, -345.2850424684869495 ) ) ;
#44000=CARTESIAN_POINT ( 'NONE',  ( 30.03678288590383261, -295.3722993304892270, -299.9502197308556219 ) ) ;
#44002=CARTESIAN_POINT ( 'NONE',  ( -90.51758653591971893, -296.6320981476472980, -320.6827151364626047 ) ) ;
#44003=DIRECTION ( 'NONE',  ( -5.501794166262391869E-14, -0.01273136352371387336, 0.9999189529070978688 ) ) ;
#44004=CARTESIAN_POINT ( 'NONE',  ( -103.9658304673356781, -283.0380823914529742, -235.0410544692495023 ) ) ;
#44005=CARTESIAN_POINT ( 'NONE',  ( -108.5918691158734362, -296.3425693358669832, -286.2486419939053235 ) ) ;
#44006=CARTESIAN_POINT ( 'NONE',  ( -96.27031319143111432, -283.8845804630171301, -319.9437883758359362 ) ) ;
#44007=CARTESIAN_POINT ( 'NONE',  ( -37.29021556066937393, -284.9716242599978955, -345.9339257643217138 ) ) ;
#44008=CARTESIAN_POINT ( 'NONE',  ( 34.83587874115121963, -286.8804463637044364, -243.6002996086376413 ) ) ;
#44009=CARTESIAN_POINT ( 'NONE',  ( 37.47377772135444474, -291.5935751655678132, -273.5929287683359235 ) ) ;
#44010=CARTESIAN_POINT ( 'NONE',  ( -111.9267015750301368, -277.9815159672648406, -251.8345809438482092 ) ) ;
#44011=CARTESIAN_POINT ( 'NONE',  ( -106.6379572354042153, -270.4809262143061233, -236.9535640164627068 ) ) ;
#44013=CARTESIAN_POINT ( 'NONE',  ( 18.97625804578514064, -285.6824366292649415, -223.2733042783450799 ) ) ;
#44014=CARTESIAN_POINT ( 'NONE',  ( -114.0592620446531384, -289.4977473901165013, -268.3490466277049222 ) ) ;
#44016=CARTESIAN_POINT ( 'NONE',  ( -95.39020467250708180, -297.5165932479951039, -315.9331657504804980 ) ) ;
#44017=CARTESIAN_POINT ( 'NONE',  ( -99.77807564016275421, -280.5647437018456571, -226.3122212162727749 ) ) ;
#44018=CARTESIAN_POINT ( 'NONE',  ( 31.89513393361116655, -291.9609026510638046, -300.2361549402726268 ) ) ;
#44019=CARTESIAN_POINT ( 'NONE',  ( 35.16024665971853835, -281.3389308217348344, -279.4650824045208992 ) ) ;
#44020=CARTESIAN_POINT ( 'NONE',  ( -66.92247652897121668, -295.5959084278559317, -341.4666527624883656 ) ) ;
#44021=CARTESIAN_POINT ( 'NONE',  ( 27.47609378644173361, -285.1147926927037588, -231.4275956051534422 ) ) ;
#44022=CARTESIAN_POINT ( 'NONE',  ( -111.7779455287604549, -280.4291977328733765, -279.9497437665503980 ) ) ;
#44023=CARTESIAN_POINT ( 'NONE',  ( -109.9679735975299479, -295.7398603426686918, -260.5533841559553707 ) ) ;
#44026=CARTESIAN_POINT ( 'NONE',  ( 37.34895488333177838, -283.5442926905524246, -271.3100599552428207 ) ) ;
#44028=CARTESIAN_POINT ( 'NONE',  ( -106.6379572354042296, -294.4809262143061233, -236.9535640164627353 ) ) ;
#44029=CARTESIAN_POINT ( 'NONE',  ( 13.86449909642468903, -273.9457036916368224, -213.0005312680847283 ) ) ;
#44030=CARTESIAN_POINT ( 'NONE',  ( -90.75773791819591452, -291.1010935544093172, -220.5859595276169784 ) ) ;
#44031=CARTESIAN_POINT ( 'NONE',  ( 30.98454119687911756, -283.4385049435863948, -297.9696763904863701 ) ) ;
#44032=CARTESIAN_POINT ( 'NONE',  ( -85.85118687162413664, -274.9675836832465734, -214.6758155856233543 ) ) ;
#44033=CARTESIAN_POINT ( 'NONE',  ( -24.64658907743955751, -284.4930211980681065, -345.5497161803204449 ) ) ;
#44034=CARTESIAN_POINT ( 'NONE',  ( 33.70401374697776475, -280.5896469540128919, -288.8403828828775204 ) ) ;
#44035=CARTESIAN_POINT ( 'NONE',  ( -99.66950811787887687, -281.1173109069549696, -228.5526125903427612 ) ) ;
#44036=CARTESIAN_POINT ( 'NONE',  ( 30.78831685937531049, -298.8830859118043577, -193.3610866696328685 ) ) ;
#44038=CARTESIAN_POINT ( 'NONE',  ( -71.40089124612519811, -273.4480738680367722, -201.3033776132195669 ) ) ;
#44039=CARTESIAN_POINT ( 'NONE',  ( 33.15705719761975701, -295.1590049182086659, -246.3001998660506899 ) ) ;
#44043=CARTESIAN_POINT ( 'NONE',  ( 27.04354491183867637, -292.2236898665133253, -310.3951552170983064 ) ) ;
#44044=CARTESIAN_POINT ( 'NONE',  ( -51.56730856098430849, -273.3730523486319157, -198.6460418883233672 ) ) ;
#44046=CARTESIAN_POINT ( 'NONE',  ( -73.12586384935194417, -293.1067565478068104, -202.9504948871793317 ) ) ;
#44047=CARTESIAN_POINT ( 'NONE',  ( 35.77081079830085031, -283.8376638359844719, -253.6410175316879361 ) ) ;
#44048=CARTESIAN_POINT ( 'NONE',  ( 10.85697776918869550, -293.9066046520351847, -210.7538535782440192 ) ) ;
#44049=CARTESIAN_POINT ( 'NONE',  ( 21.82221221409689704, -290.1820178877637204, -316.2039214950164023 ) ) ;
#44050=CARTESIAN_POINT ( 'NONE',  ( 21.44729925277438198, -274.1893918510941717, -316.6838195015088218 ) ) ;
#44051=CARTESIAN_POINT ( 'NONE',  ( -62.24905186942313406, -279.2986389848290969, -340.5653095155972210 ) ) ;
#44052=CARTESIAN_POINT ( 'NONE',  ( 17.19785535431074663, -292.3461535648852987, -321.0242316466182615 ) ) ;
#44053=CARTESIAN_POINT ( 'NONE',  ( 10.03191374539644443, -282.5570908980043328, -211.1665178621244365 ) ) ;
#44055=CARTESIAN_POINT ( 'NONE',  ( -36.19745628623380185, -282.7041319216452280, -343.3732963701150425 ) ) ;
#44056=CARTESIAN_POINT ( 'NONE',  ( -90.85237773420880103, -280.3943191650643030, -215.3498351192494624 ) ) ;
#44057=CARTESIAN_POINT ( 'NONE',  ( 33.19427606454001989, -280.7308528344065621, -300.3743469823941723 ) ) ;
#44058=CARTESIAN_POINT ( 'NONE',  ( 0.9401287792214468864, -277.4959810107822022, -336.9595388358503101 ) ) ;
#44060=CARTESIAN_POINT ( 'NONE',  ( 14.42714466803189488, -277.8602959427839778, -326.4927907685060973 ) ) ;
#44061=CARTESIAN_POINT ( 'NONE',  ( -82.08285599513421005, -292.1948066931273615, -326.5171145203363494 ) ) ;
#44063=CARTESIAN_POINT ( 'NONE',  ( -112.1759815451095648, -274.5879229915463497, -267.5942600973444314 ) ) ;
#44064=CARTESIAN_POINT ( 'NONE',  ( -35.09278364630892355, -275.0438771422349760, -344.9720366219190169 ) ) ;
#44065=CARTESIAN_POINT ( 'NONE',  ( -112.1318886583186298, -292.1411412107378851, -283.8658639234906786 ) ) ;
#44066=CARTESIAN_POINT ( 'NONE',  ( 21.40344152879438866, -293.5099179007456769, -313.8686000995709833 ) ) ;
#44067=CARTESIAN_POINT ( 'NONE',  ( 21.43794956855026257, -287.7291601388004665, -320.0046440960488212 ) ) ;
#44068=CARTESIAN_POINT ( 'NONE',  ( -32.07140973467762990, -293.5616551262005487, -346.6030736061757693 ) ) ;
#44069=CARTESIAN_POINT ( 'NONE',  ( -48.46919692003073266, -281.5960250828873086, -343.3174009800020485 ) ) ;
#44070=CARTESIAN_POINT ( 'NONE',  ( -37.24298847226193487, -290.9113190842841163, -344.5962561593825626 ) ) ;
#44071=CARTESIAN_POINT ( 'NONE',  ( -110.1867015026350600, -282.8820420828877218, -281.8386576080146142 ) ) ;
#44072=CARTESIAN_POINT ( 'NONE',  ( -51.09386472680689195, -284.5466457170364265, -342.6080647163242929 ) ) ;
#44073=CARTESIAN_POINT ( 'NONE',  ( -95.27283547468262270, -290.8104941890112514, -320.7278110533723634 ) ) ;
#44074=CARTESIAN_POINT ( 'NONE',  ( 35.76448144918371241, -282.0569870537689212, -271.3083043585982068 ) ) ;
#44075=CARTESIAN_POINT ( 'NONE',  ( -50.48307129441754881, -290.6828405046820762, -194.8938198896414065 ) ) ;
#44076=CARTESIAN_POINT ( 'NONE',  ( -30.90758565753862896, -286.9343125435161710, -193.7791826253577483 ) ) ;
#44077=CARTESIAN_POINT ( 'NONE',  ( 38.04924404560624396, -288.2366681199042660, -285.7146986745073036 ) ) ;
#44078=CARTESIAN_POINT ( 'NONE',  ( -38.62703663849384839, -286.2023055395117694, -197.3599528656638711 ) ) ;
#44079=ORIENTED_EDGE ( 'NONE', *, *, #60023, .T. ) ;
#44081=CARTESIAN_POINT ( 'NONE',  ( 1.162439852943140117, -296.4041810372761461, -335.6124527175344383 ) ) ;
#44082=CARTESIAN_POINT ( 'NONE',  ( -41.93281779182947133, -293.7935620943900403, -346.7821476352028185 ) ) ;
#44083=CARTESIAN_POINT ( 'NONE',  ( -94.64461489327443644, -276.9687349921433679, -315.9858064458254034 ) ) ;
#44084=CARTESIAN_POINT ( 'NONE',  ( -40.42784804039752089, -297.3630355600913617, -193.4729457260481240 ) ) ;
#44085=CARTESIAN_POINT ( 'NONE',  ( 35.00134795276837707, -292.2155278483286338, -284.4035945560945606 ) ) ;
#44086=CARTESIAN_POINT ( 'NONE',  ( 1.120180119018857390, -276.3334292749432279, -207.1261768427396532 ) ) ;
#44087=CARTESIAN_POINT ( 'NONE',  ( -100.7535733172028074, -295.3112091459133808, -232.0920309628987184 ) ) ;
#44088=CARTESIAN_POINT ( 'NONE',  ( 34.16574114520963690, -294.9749937863874720, -286.9639354778252027 ) ) ;
#44089=CARTESIAN_POINT ( 'NONE',  ( 32.08937811181002076, -294.3186577444822092, -246.6755098941000597 ) ) ;
#44091=CARTESIAN_POINT ( 'NONE',  ( -104.3355556495353085, -294.1010451522216158, -304.5617979576796870 ) ) ;
#44092=CARTESIAN_POINT ( 'NONE',  ( -69.15345023634576194, -275.6339466818183155, -202.4278764260954802 ) ) ;
#44093=CARTESIAN_POINT ( 'NONE',  ( -108.9431327409230335, -291.6956845764705690, -254.9779032123171021 ) ) ;
#44094=CARTESIAN_POINT ( 'NONE',  ( -58.41028401930568492, -295.6654315039409653, -340.2767976225544544 ) ) ;
#44095=CARTESIAN_POINT ( 'NONE',  ( -102.1774678322762355, -280.0196401391015115, -308.8656015513670923 ) ) ;
#44096=CARTESIAN_POINT ( 'NONE',  ( -84.25126708559081123, -278.1073271894395589, -209.8557645281158841 ) ) ;
#44098=CARTESIAN_POINT ( 'NONE',  ( 23.43237999708655650, -275.5309273536360593, -317.4974788400439820 ) ) ;
#44099=CARTESIAN_POINT ( 'NONE',  ( -111.3064047064652016, -282.5175766163941375, -279.2056421071889645 ) ) ;
#44100=CARTESIAN_POINT ( 'NONE',  ( -112.2063405631591593, -277.1324029294298157, -256.0884034393978936 ) ) ;
#44101=CARTESIAN_POINT ( 'NONE',  ( -67.90322790702578004, -277.6518030891620583, -201.6737823018166580 ) ) ;
#44103=CARTESIAN_POINT ( 'NONE',  ( -110.7754166671343086, -271.1989731141462698, -264.8514040384455370 ) ) ;
#44104=CARTESIAN_POINT ( 'NONE',  ( -1.849681332598452244, -276.5224153657350712, -204.2762730632705370 ) ) ;
#44107=CARTESIAN_POINT ( 'NONE',  ( -72.64043411783150361, -289.6073080689881749, -203.7702201917964828 ) ) ;
#44109=CARTESIAN_POINT ( 'NONE',  ( -78.13640619104597818, -289.5841849134964718, -335.7286898721372381 ) ) ;
#44110=CARTESIAN_POINT ( 'NONE',  ( -36.97488297297677917, -276.0569231675438004, -195.1826011640731053 ) ) ;
#44111=CARTESIAN_POINT ( 'NONE',  ( -36.43070675429654415, -296.0634240084475550, -195.5280873641150663 ) ) ;
#44112=CARTESIAN_POINT ( 'NONE',  ( -80.83835934114465260, -284.6757198884120612, -206.9549748846036437 ) ) ;
#44115=CARTESIAN_POINT ( 'NONE',  ( -104.0717042862764288, -282.0978181708819648, -304.7093259955146323 ) ) ;
#44117=CARTESIAN_POINT ( 'NONE',  ( -5.857461145425837401, -291.2704756189223758, -204.0458778779909892 ) ) ;
#44118=CARTESIAN_POINT ( 'NONE',  ( -109.8666489912981916, -282.8980214791935737, -254.4589625155815895 ) ) ;
#44119=DIRECTION ( 'NONE',  ( 0.9999189529070979798, -0.01273136352371030157, 0.000000000000000000 ) ) ;
#44120=CARTESIAN_POINT ( 'NONE',  ( 31.70674536624019879, -291.1678279935823639, -240.9482378215590472 ) ) ;
#44121=CARTESIAN_POINT ( 'NONE',  ( -70.79745113023881231, -279.1012749278464184, -336.1422181713911073 ) ) ;
#44122=CARTESIAN_POINT ( 'NONE',  ( -93.63840408274512583, -286.4688374217048477, -218.3344450476159864 ) ) ;
#44123=CARTESIAN_POINT ( 'NONE',  ( 34.68249033531274961, -273.9246005445561991, -293.2047207221085614 ) ) ;
#44124=CARTESIAN_POINT ( 'NONE',  ( -38.62490764333821858, -286.0356524706753589, -197.3599154069878239 ) ) ;
#44125=CARTESIAN_POINT ( 'NONE',  ( -108.7393801580826818, -279.7434630676462461, -288.2384494771071672 ) ) ;
#44126=CARTESIAN_POINT ( 'NONE',  ( -16.32472344052246882, -277.5764120391957590, -340.4919777814241684 ) ) ;
#44127=CARTESIAN_POINT ( 'NONE',  ( -99.35748562819151175, -287.1243932113331425, -228.0906294698411614 ) ) ;
#44129=CARTESIAN_POINT ( 'NONE',  ( -110.6395504398199847, -271.5021483123970825, -270.3477634379551660 ) ) ;
#44130=CARTESIAN_POINT ( 'NONE',  ( -112.8882716364605159, -296.5725423155080307, -255.4032052554253198 ) ) ;
#44131=CARTESIAN_POINT ( 'NONE',  ( 19.08509719053820675, -290.2137259213678817, -319.3043090022773640 ) ) ;
#44133=CARTESIAN_POINT ( 'NONE',  ( 13.84574458161073096, -278.9090924074131408, -334.4957818155094174 ) ) ;
#44134=CARTESIAN_POINT ( 'NONE',  ( -92.84052196834250026, -278.1997472452241027, -217.3572569169104440 ) ) ;
#44135=CARTESIAN_POINT ( 'NONE',  ( 16.93424471673715814, -291.2091459564875322, -216.8025723418089115 ) ) ;
#44136=CARTESIAN_POINT ( 'NONE',  ( 35.81481182980429168, -289.1883037335769586, -279.2398853642694121 ) ) ;
#44137=CARTESIAN_POINT ( 'NONE',  ( -46.60520626743090133, -281.6932587640106362, -196.8779665232102616 ) ) ;
#44138=CARTESIAN_POINT ( 'NONE',  ( 16.28545371658437801, -289.7344440529325311, -324.8657211449441320 ) ) ;
#44139=CARTESIAN_POINT ( 'NONE',  ( -108.4361152196800333, -286.8630330684059118, -246.3114162501495628 ) ) ;
#44140=CARTESIAN_POINT ( 'NONE',  ( -70.29909077224183989, -277.6411918085017874, -339.9658592409560356 ) ) ;
#44141=VERTEX_POINT ( 'NONE', #47621 ) ;
#44142=CARTESIAN_POINT ( 'NONE',  ( -110.9278836594412496, -270.7306310512091727, -256.4792130527324616 ) ) ;
#44143=CARTESIAN_POINT ( 'NONE',  ( 37.43061990652664406, -291.4888294980463570, -259.1274482269715236 ) ) ;
#44144=CARTESIAN_POINT ( 'NONE',  ( -35.33390146101689311, -279.9099900183558702, -193.3741626031550709 ) ) ;
#44145=CARTESIAN_POINT ( 'NONE',  ( -59.87271460015958979, -275.6176736148978534, -199.5738591962133910 ) ) ;
#44147=CARTESIAN_POINT ( 'NONE',  ( -37.30987171927208124, -291.5519495502701943, -345.3611179825600175 ) ) ;
#44148=CARTESIAN_POINT ( 'NONE',  ( -36.92251312779276873, -272.2972305803796189, -194.3627234916388602 ) ) ;
#44150=CARTESIAN_POINT ( 'NONE',  ( -30.25017641578499195, -279.6517930434106916, -197.5941559951730255 ) ) ;
#44151=CARTESIAN_POINT ( 'NONE',  ( -2.889871793493798524, -277.8121324800636671, -338.7941418375052081 ) ) ;
#44152=CARTESIAN_POINT ( 'NONE',  ( -92.29691102077217124, -298.6716372440093323, -221.4193187341389546 ) ) ;
#44153=CARTESIAN_POINT ( 'NONE',  ( -97.86632649394189798, -282.9780834495130648, -317.5796505446180049 ) ) ;
#44154=CARTESIAN_POINT ( 'NONE',  ( 33.28728010440637064, -289.6035135905833044, -292.6569862521859022 ) ) ;
#44155=CARTESIAN_POINT ( 'NONE',  ( -108.2515440643995674, -298.4346764019963416, -242.0321233671757852 ) ) ;
#44157=CARTESIAN_POINT ( 'NONE',  ( -89.35003785156875722, -298.5445892839471185, -214.0474356187960154 ) ) ;
#44159=CARTESIAN_POINT ( 'NONE',  ( 33.27843931474874495, -295.8754012364652795, -295.2717191445337903 ) ) ;
#44160=CARTESIAN_POINT ( 'NONE',  ( -88.19285662459073194, -281.7653921851065206, -325.3336579998240268 ) ) ;
#44161=CARTESIAN_POINT ( 'NONE',  ( -88.44132444995396725, -271.3522266511541829, -215.8782857808451467 ) ) ;
#44162=CARTESIAN_POINT ( 'NONE',  ( 35.08223714319956343, -288.8491702274219506, -246.5025610590157044 ) ) ;
#44163=CARTESIAN_POINT ( 'NONE',  ( -45.41006640045394960, -288.0771063677282768, -343.2248781042105179 ) ) ;
#44164=CARTESIAN_POINT ( 'NONE',  ( 195.5582280236794475, 277.9486174577299380, -125.6969904412313070 ) ) ;
#44166=CARTESIAN_POINT ( 'NONE',  ( -38.92629107760777885, -287.6464015149084048, -346.7554591757346998 ) ) ;
#44167=CARTESIAN_POINT ( 'NONE',  ( -69.98571976429278152, -289.1611452922231820, -335.6930913783895107 ) ) ;
#44169=CARTESIAN_POINT ( 'NONE',  ( -46.48234764152076792, -287.0183941167695139, -194.2169056462059871 ) ) ;
#44170=CARTESIAN_POINT ( 'NONE',  ( -7.495127165695278038, -276.9829737251915844, -337.0039688313361808 ) ) ;
#44171=CARTESIAN_POINT ( 'NONE',  ( 3.986582512691288382, -291.5148054197242686, -205.6957994855593483 ) ) ;
#44172=CARTESIAN_POINT ( 'NONE',  ( -0.4170870768949739293, -283.2259664171843383, -337.8288788632528963 ) ) ;
#44173=CARTESIAN_POINT ( 'NONE',  ( -2.722154013542533502, -282.0215261930935071, -202.3450922761558672 ) ) ;
#44174=CARTESIAN_POINT ( 'NONE',  ( -74.26211103376897427, -283.8620768005749255, -337.9678166649973718 ) ) ;
#44175=CARTESIAN_POINT ( 'NONE',  ( 32.75369649040284514, -281.6148138787478388, -249.8983992065044220 ) ) ;
#44176=CARTESIAN_POINT ( 'NONE',  ( 154.0998481207909379, 207.0352699179129559, -217.4206707551776105 ) ) ;
#44178=CARTESIAN_POINT ( 'NONE',  ( -70.02980485779180242, -279.4838224125497845, -337.6918383107881709 ) ) ;
#44179=CARTESIAN_POINT ( 'NONE',  ( 24.23470416219412371, -22.50377800736068323, -344.3197070345564725 ) ) ;
#44180=CARTESIAN_POINT ( 'NONE',  ( 201.0615436985592908, 293.2992059325864034, -68.27523266910206701 ) ) ;
#44182=CARTESIAN_POINT ( 'NONE',  ( -104.5239402591454478, -272.1392627428297146, -241.2647166030098163 ) ) ;
#44183=CARTESIAN_POINT ( 'NONE',  ( 38.00904969897577956, -293.2544328439536230, -285.9107611931934798 ) ) ;
#44184=CARTESIAN_POINT ( 'NONE',  ( 174.2662291550402074, 240.3192241394675079, -177.2675829000265537 ) ) ;
#44186=CARTESIAN_POINT ( 'NONE',  ( -99.15862868464212454, -271.8401489300471781, -225.1959667016525373 ) ) ;
#44187=CARTESIAN_POINT ( 'NONE',  ( -110.9219885117268234, -288.8695857362028505, -276.6783256055854281 ) ) ;
#44188=CARTESIAN_POINT ( 'NONE',  ( -78.61717904793809453, -297.4744966252449103, -332.1257089985984408 ) ) ;
#44189=CARTESIAN_POINT ( 'NONE',  ( 23.16536800631423532, -289.4446340011258485, -312.0982709022560471 ) ) ;
#44191=CARTESIAN_POINT ( 'NONE',  ( -88.43984633436494391, -296.6887950310547808, -327.7193832130890883 ) ) ;
#44193=CARTESIAN_POINT ( 'NONE',  ( 18.70493752357450035, -287.3795849803549913, -223.4719925560505658 ) ) ;
#44194=CARTESIAN_POINT ( 'NONE',  ( -106.5583079042602037, -271.8975530742450246, -237.3375852092785863 ) ) ;
#44195=CARTESIAN_POINT ( 'NONE',  ( 23.05111624384964841, -294.9918123902675688, -317.8887209517366159 ) ) ;
#44196=CARTESIAN_POINT ( 'NONE',  ( 39.54561512865520001, -294.0796059905883340, -273.1660521483253206 ) ) ;
#44197=CARTESIAN_POINT ( 'NONE',  ( -62.80271767970420171, -291.8779247651003743, -201.9452090889473368 ) ) ;
#44198=EDGE_LOOP ( 'NONE', ( #30349, #79293 ) ) ;
#44199=CARTESIAN_POINT ( 'NONE',  ( -70.78781701246508362, -275.5345701890504984, -202.6066239058280019 ) ) ;
#44200=CARTESIAN_POINT ( 'NONE',  ( 36.49874880616503248, -274.6043469331105484, -290.7961831706880957 ) ) ;
#44202=CARTESIAN_POINT ( 'NONE',  ( -94.91157564584894146, -278.7519079637411323, -219.3196021724193088 ) ) ;
#44203=CARTESIAN_POINT ( 'NONE',  ( 33.27602869215502324, -274.2333270949336566, -291.8426268657913738 ) ) ;
#44204=CARTESIAN_POINT ( 'NONE',  ( -59.58245494610068249, -274.8370548186397286, -200.4540145010778929 ) ) ;
#44205=CARTESIAN_POINT ( 'NONE',  ( -56.93606160809189021, -274.7345605476013475, -199.7428733336180358 ) ) ;
#44206=CARTESIAN_POINT ( 'NONE',  ( -82.98948492906988861, -275.1976673495402679, -209.5477897017458133 ) ) ;
#44207=CARTESIAN_POINT ( 'NONE',  ( 35.01380846795892410, -273.3004200898033105, -249.1289194178671949 ) ) ;
#44208=CARTESIAN_POINT ( 'NONE',  ( -42.38849250033216975, -295.7688954099421608, -343.2886337433527615 ) ) ;
#44209=CARTESIAN_POINT ( 'NONE',  ( 12.74272004544800296, -292.9120683986142808, -324.3468572826103582 ) ) ;
#44211=CARTESIAN_POINT ( 'NONE',  ( 3.474174293229708166, -277.0116810888953296, -335.6433970705903675 ) ) ;
#44212=CARTESIAN_POINT ( 'NONE',  ( -46.18088475194703335, -274.1035764587128938, -197.8982390742496023 ) ) ;
#44213=CARTESIAN_POINT ( 'NONE',  ( -108.5632250512156247, -283.5951063048372589, -242.2744572681871773 ) ) ;
#44214=CARTESIAN_POINT ( 'NONE',  ( -96.80805936358210317, -297.9236062943652996, -316.3369871953059942 ) ) ;
#44216=CARTESIAN_POINT ( 'NONE',  ( -98.23581421593654284, -284.3110344478233174, -229.8085767988599741 ) ) ;
#44217=CARTESIAN_POINT ( 'NONE',  ( -110.0428307851742034, -276.6106056074396520, -284.3033307366886220 ) ) ;
#44218=CARTESIAN_POINT ( 'NONE',  ( -91.41303848245777885, -276.4150650546976067, -320.3518441923130808 ) ) ;
#44219=CARTESIAN_POINT ( 'NONE',  ( -110.4719326398463863, -286.7667217879182999, -253.6621375893454058 ) ) ;
#44220=CARTESIAN_POINT ( 'NONE',  ( 15.72331339533422678, -276.0290172102775159, -219.5802184918402986 ) ) ;
#44222=CARTESIAN_POINT ( 'NONE',  ( 23.84974165440123173, -273.3419448418790694, -224.9513407345810947 ) ) ;
#44223=CARTESIAN_POINT ( 'NONE',  ( -94.52800328201561797, -281.2264783127059218, -221.5586059181094924 ) ) ;
#44225=CARTESIAN_POINT ( 'NONE',  ( -64.06128927176088439, -287.6265035753560255, -199.6692269937903461 ) ) ;
#44227=CARTESIAN_POINT ( 'NONE',  ( 15.23539413068917270, -290.7939003430067260, -216.8047613663628681 ) ) ;
#44228=EDGE_CURVE ( 'NONE', #47701, #75524, #55639, .T. ) ;
#44230=CARTESIAN_POINT ( 'NONE',  ( -82.17459559740092345, -296.2202369010653911, -212.1835314915800268 ) ) ;
#44231=CARTESIAN_POINT ( 'NONE',  ( -75.59615210149343056, -289.6759379042433125, -206.6814448480564863 ) ) ;
#44232=CARTESIAN_POINT ( 'NONE',  ( -107.3349855510151656, -256.5393008024622077, -313.9713749062190686 ) ) ;
#44233=FACE_OUTER_BOUND ( 'NONE', #68617, .T. ) ;
#44234=CARTESIAN_POINT ( 'NONE',  ( -101.7267520673037922, -288.4892405297173354, -311.4129121200614918 ) ) ;
#44235=CARTESIAN_POINT ( 'NONE',  ( 16.42250400512222797, -283.8728382227190536, -320.9902921522305519 ) ) ;
#44236=CARTESIAN_POINT ( 'NONE',  ( -110.7365007942342885, -283.0439403702375216, -250.4867607419369335 ) ) ;
#44237=CARTESIAN_POINT ( 'NONE',  ( 16.26746647612966612, -283.6980103413923757, -320.8472754617042710 ) ) ;
#44238=CARTESIAN_POINT ( 'NONE',  ( -96.04520858568972130, -284.7438653608107870, -314.0246018351343764 ) ) ;
#44239=CARTESIAN_POINT ( 'NONE',  ( -109.9502291657798452, -292.2739538444660639, -290.5206893010515046 ) ) ;
#44241=CARTESIAN_POINT ( 'NONE',  ( -31.26596745729547067, -274.4601643074283857, -193.6091292834974524 ) ) ;
#44243=CARTESIAN_POINT ( 'NONE',  ( 7.068035009423874193, -286.5329084905408763, -331.5573651096770504 ) ) ;
#44244=CARTESIAN_POINT ( 'NONE',  ( 26.14456769441573414, -274.9768540199766562, -226.7660392318886977 ) ) ;
#44245=CARTESIAN_POINT ( 'NONE',  ( 37.35404291076277161, -295.5369866900414877, -270.7437446896001347 ) ) ;
#44247=CARTESIAN_POINT ( 'NONE',  ( -106.6662871844225293, -293.4805209788415823, -237.0123917617630980 ) ) ;
#44248=CARTESIAN_POINT ( 'NONE',  ( -26.68772616763157046, -281.5987579708564112, -343.1295855098389893 ) ) ;
#44250=CARTESIAN_POINT ( 'NONE',  ( -108.9286662694375138, -276.2548504243796970, -293.4490655206435008 ) ) ;
#44251=CARTESIAN_POINT ( 'NONE',  ( -94.55370034198027440, -271.7219805740683682, -219.8685959108111092 ) ) ;
#44252=CARTESIAN_POINT ( 'NONE',  ( 7.636591263180227074, -275.7684751826718070, -328.0523955772432032 ) ) ;
#44254=CARTESIAN_POINT ( 'NONE',  ( -68.10813376321992507, -293.1607865170478249, -203.3835721314831915 ) ) ;
#44256=CARTESIAN_POINT ( 'NONE',  ( 11.07741701989542449, -293.6830193049062814, -215.3480533558231684 ) ) ;
#44257=CARTESIAN_POINT ( 'NONE',  ( -110.1944039448576405, -286.4830971900316854, -257.2337614647697706 ) ) ;
#44258=CARTESIAN_POINT ( 'NONE',  ( 10.73386698722642407, -294.1267657837903471, -210.9015922608761002 ) ) ;
#44259=CARTESIAN_POINT ( 'NONE',  ( 39.01122901738659010, -294.9381259910376798, -275.9860984305571492 ) ) ;
#44260=CARTESIAN_POINT ( 'NONE',  ( -92.19207784247504378, -295.6978372760135017, -318.5320227810769893 ) ) ;
#44261=CARTESIAN_POINT ( 'NONE',  ( -56.55399730580961659, -291.2998115424617254, -342.9126154468874574 ) ) ;
#44262=CARTESIAN_POINT ( 'NONE',  ( -98.04311187050015519, -284.0858361666709015, -317.7355690824039129 ) ) ;
#44263=CARTESIAN_POINT ( 'NONE',  ( -112.3183849281744244, -270.8348142488693497, -259.1044052736238541 ) ) ;
#44264=CARTESIAN_POINT ( 'NONE',  ( -99.34297766170321609, -284.9930855666974594, -224.6133253961504010 ) ) ;
#44265=CARTESIAN_POINT ( 'NONE',  ( -81.77879077782938566, -279.6406875791032007, -330.3377115366125736 ) ) ;
#44266=CARTESIAN_POINT ( 'NONE',  ( -109.0495640668344492, -283.5532556106758761, -254.6464188711234442 ) ) ;
#44267=CARTESIAN_POINT ( 'NONE',  ( 15.26448937178230558, -286.3095632037154701, -323.8897361082658790 ) ) ;
#44268=CARTESIAN_POINT ( 'NONE',  ( -107.3619393009930150, -277.0655587574885885, -241.4220166775552343 ) ) ;
#44271=CARTESIAN_POINT ( 'NONE',  ( -109.2524821411010549, -284.2309727311548500, -257.3745831739649361 ) ) ;
#44272=CARTESIAN_POINT ( 'NONE',  ( 5.947164010663343880, -281.8301973971152847, -207.1623604055843941 ) ) ;
#44273=CARTESIAN_POINT ( 'NONE',  ( -74.32451217551619038, -288.5902225194246284, -337.6449293966938967 ) ) ;
#44274=CARTESIAN_POINT ( 'NONE',  ( -64.78770275756014030, -279.0046608303928792, -341.5023758337149502 ) ) ;
#44276=CARTESIAN_POINT ( 'NONE',  ( -98.39967108264154660, -279.2491628226472358, -316.4827487892523550 ) ) ;
#44277=CARTESIAN_POINT ( 'NONE',  ( -9.245385095142074405, -280.2633230881125996, -202.9845858212300413 ) ) ;
#44279=CARTESIAN_POINT ( 'NONE',  ( 10.52084277501579912, -276.6963827057916205, -213.0132279692040242 ) ) ;
#44280=CARTESIAN_POINT ( 'NONE',  ( 38.35725277512000275, -293.7293203700261870, -284.5273437214487444 ) ) ;
#44281=CARTESIAN_POINT ( 'NONE',  ( -31.77326406589785890, -287.0017718883546536, -344.8496958323131025 ) ) ;
#44282=CARTESIAN_POINT ( 'NONE',  ( -81.48370377214789073, -293.0626865193349886, -208.2489297427242434 ) ) ;
#44283=AXIS2_PLACEMENT_3D ( 'NONE', #10015, #30408, #31804 ) ;
#44284=CARTESIAN_POINT ( 'NONE',  ( -66.18737576575108505, -294.3591806187856719, -337.7566153932162933 ) ) ;
#44285=CARTESIAN_POINT ( 'NONE',  ( 30.60367693512107934, -293.5781292341820290, -297.2485209610801462 ) ) ;
#44286=CARTESIAN_POINT ( 'NONE',  ( -98.11178808324184786, -292.2587806512038924, -223.5585752111180113 ) ) ;
#44287=CARTESIAN_POINT ( 'NONE',  ( 30.43213151035883257, -282.5699360638055282, -297.7582056555559689 ) ) ;
#44288=CARTESIAN_POINT ( 'NONE',  ( -113.3096713220419787, -271.7538298802033410, -258.9677402597746436 ) ) ;
#44289=CARTESIAN_POINT ( 'NONE',  ( -48.84554408078385990, -289.8462754519599116, -346.4477091772499193 ) ) ;
#44290=CARTESIAN_POINT ( 'NONE',  ( -67.41323597047463068, -281.5819763459932688, -339.9025316476034959 ) ) ;
#44291=CARTESIAN_POINT ( 'NONE',  ( 31.67034875309768793, -288.3251596649110979, -304.5853281146143559 ) ) ;
#44292=CARTESIAN_POINT ( 'NONE',  ( -91.53976564075794897, -285.5867395296721725, -221.3515810274289493 ) ) ;
#44293=CARTESIAN_POINT ( 'NONE',  ( 202.9738562182569694, 295.9636489450776367, -54.00000000004089173 ) ) ;
#44294=CARTESIAN_POINT ( 'NONE',  ( -72.20741897415064159, -195.2005351582145920, -358.5414825501330824 ) ) ;
#44295=CARTESIAN_POINT ( 'NONE',  ( -47.44010110492147447, -155.2456545128756886, -361.2982599994518864 ) ) ;
#44296=CARTESIAN_POINT ( 'NONE',  ( -91.40927597213088518, -278.4545472724033743, -221.0731988796577809 ) ) ;
#44297=CARTESIAN_POINT ( 'NONE',  ( -91.20427172815162464, -276.7606101788438764, -320.1647378175440508 ) ) ;
#44298=CARTESIAN_POINT ( 'NONE',  ( -10.35105033397390883, -274.0615003983485849, -198.2124598010597936 ) ) ;
#44299=CARTESIAN_POINT ( 'NONE',  ( 86.02760830248789148, 81.15136696978881048, -299.6155979961977209 ) ) ;
#44300=CARTESIAN_POINT ( 'NONE',  ( -111.1570698369404653, -277.3766041890256702, -250.5648273664892827 ) ) ;
#44301=CARTESIAN_POINT ( 'NONE',  ( -2.884028679770540560, -280.6145789443700096, -336.5911121559167896 ) ) ;
#44302=CARTESIAN_POINT ( 'NONE',  ( -37.66191096783632730, -296.8162085151935230, -346.3600199473525549 ) ) ;
#44303=CARTESIAN_POINT ( 'NONE',  ( -1.231711286763641722, -293.0373959675957849, -206.8324032252917846 ) ) ;
#44304=CARTESIAN_POINT ( 'NONE',  ( -60.81062250351171627, -274.6962675792217397, -197.2164631965916612 ) ) ;
#44305=CARTESIAN_POINT ( 'NONE',  ( -37.28433474693761696, -287.7362434404299734, -343.8542481986509642 ) ) ;
#44306=CARTESIAN_POINT ( 'NONE',  ( -35.83594424014573576, -298.5628754214549190, -193.4225339918467625 ) ) ;
#44307=CARTESIAN_POINT ( 'NONE',  ( -109.3625686777309198, -296.5616392050403647, -282.2772624038217373 ) ) ;
#44310=ADVANCED_FACE ( 'NONE', ( #42864 ), #32519, .T. ) ;
#44311=CARTESIAN_POINT ( 'NONE',  ( -110.7698943111320915, -280.2444763586340741, -288.2369826619550395 ) ) ;
#44314=CARTESIAN_POINT ( 'NONE',  ( -9.141089901701752396, -281.5094732023418942, -202.6931665065401944 ) ) ;
#44315=CARTESIAN_POINT ( 'NONE',  ( -81.93327532074388841, -279.4108154737498921, -331.8880668207454505 ) ) ;
#44316=CARTESIAN_POINT ( 'NONE',  ( -48.96589212619218756, -272.3813992028697726, -197.5386834195107895 ) ) ;
#44319=CARTESIAN_POINT ( 'NONE',  ( -54.49484821393048861, -279.9923816359219586, -199.3528106552576276 ) ) ;
#44321=CARTESIAN_POINT ( 'NONE',  ( 38.33129238530805338, -276.1869474650199550, -256.9534359876311669 ) ) ;
#44322=CARTESIAN_POINT ( 'NONE',  ( 31.20252124061569887, -277.9511857996409390, -300.8027073419864905 ) ) ;
#44323=CARTESIAN_POINT ( 'NONE',  ( -38.55395293646709121, -275.6418077723151328, -346.7622746371741300 ) ) ;
#44326=CARTESIAN_POINT ( 'NONE',  ( -4.849709395424552483, -284.6063199712243090, -338.3655742620771321 ) ) ;
#44328=CARTESIAN_POINT ( 'NONE',  ( -47.00569737939760273, -291.1234238793411464, -197.8407147582254879 ) ) ;
#44329=CARTESIAN_POINT ( 'NONE',  ( 32.62273875463439055, -286.4908329654080035, -238.3222454954391765 ) ) ;
#44330=CARTESIAN_POINT ( 'NONE',  ( -105.0492133949513800, -282.3952231223228750, -300.2553759303422112 ) ) ;
#44331=CARTESIAN_POINT ( 'NONE',  ( -0.9764910023544955964, -281.1339448159719723, -334.3372579321289209 ) ) ;
#44332=CARTESIAN_POINT ( 'NONE',  ( 23.17627917975993412, -285.0368792986515700, -226.9280302573315851 ) ) ;
#44333=CARTESIAN_POINT ( 'NONE',  ( -62.45917585592964372, -280.9231657350135833, -201.3419456730977402 ) ) ;
#44334=CARTESIAN_POINT ( 'NONE',  ( -88.77235587117522186, -271.3304146040374007, -215.7018676450574048 ) ) ;
#44335=CARTESIAN_POINT ( 'NONE',  ( -89.90124104501845181, -282.1789037785655410, -325.6053554415149165 ) ) ;
#44336=CARTESIAN_POINT ( 'NONE',  ( -32.12550206775134853, -296.9865349872839602, -345.1924212355330042 ) ) ;
#44338=CARTESIAN_POINT ( 'NONE',  ( -103.3378633286069714, -279.0638564591805562, -302.2260956324977315 ) ) ;
#44339=CARTESIAN_POINT ( 'NONE',  ( -111.3277351600586798, -286.3786482096307964, -283.9164505795901619 ) ) ;
#44341=CARTESIAN_POINT ( 'NONE',  ( -53.11307774118312608, -293.7717778121119068, -196.4119133981878917 ) ) ;
#44343=CARTESIAN_POINT ( 'NONE',  ( -2.973054411784074702, -274.5977860903446413, -337.0229274656924758 ) ) ;
#44344=CARTESIAN_POINT ( 'NONE',  ( 22.27337497298141145, -287.4013077462379897, -318.8606999541798928 ) ) ;
#44345=CARTESIAN_POINT ( 'NONE',  ( -5.680136884807626352, -290.8754869230110103, -203.6839558843439875 ) ) ;
#44346=CARTESIAN_POINT ( 'NONE',  ( -37.82973210483599047, -275.7431786125061421, -343.8651869101385614 ) ) ;
#44347=CARTESIAN_POINT ( 'NONE',  ( -80.89834370404440733, -293.7901378483425106, -330.4750454716466948 ) ) ;
#44348=CARTESIAN_POINT ( 'NONE',  ( -86.26974549416443949, -292.6718098741879430, -215.4538438420588591 ) ) ;
#44350=DIRECTION ( 'NONE',  ( 1.000000000000000000, 0.000000000000000000, 0.000000000000000000 ) ) ;
#44351=CARTESIAN_POINT ( 'NONE',  ( -61.39157226653063759, -293.8386983675802639, -342.8339785763364489 ) ) ;
#44352=CARTESIAN_POINT ( 'NONE',  ( 18.36683560309531416, -288.4696662351336158, -221.9565782860350964 ) ) ;
#44353=CARTESIAN_POINT ( 'NONE',  ( -85.84870287679824230, -289.6312338776223783, -211.8031175765976855 ) ) ;
#44354=CARTESIAN_POINT ( 'NONE',  ( 6.207821419030736365, -289.8735238183497245, -329.7442276092970701 ) ) ;
#44355=CARTESIAN_POINT ( 'NONE',  ( 129.4467878515196162, -299.5541904835127980, -195.3611179825600175 ) ) ;
#44356=CARTESIAN_POINT ( 'NONE',  ( -72.42733682808474782, -290.3320390541636584, -334.5608050893261520 ) ) ;
#44358=CARTESIAN_POINT ( 'NONE',  ( -59.89565118516785702, -290.5431459785781954, -343.5685493637126910 ) ) ;
#44359=CARTESIAN_POINT ( 'NONE',  ( -110.4832104780518733, -276.8046467916510665, -252.1774413975929576 ) ) ;
#44360=CARTESIAN_POINT ( 'NONE',  ( -7.549092803123564011, -280.7654470216926370, -199.3669287783266668 ) ) ;
#44361=CARTESIAN_POINT ( 'NONE',  ( 6.175798002383604768, -280.2920882314238042, -206.8633097690626244 ) ) ;
#44362=CARTESIAN_POINT ( 'NONE',  ( 33.27415416238365253, -285.8794511306149388, -295.6277317301095877 ) ) ;
#44364=CARTESIAN_POINT ( 'NONE',  ( -99.00666014600341214, -277.2573572768194481, -228.9383175334328939 ) ) ;
#44365=CARTESIAN_POINT ( 'NONE',  ( -104.0181008197655217, -282.0962989754925161, -304.8148365035943357 ) ) ;
#44366=CARTESIAN_POINT ( 'NONE',  ( -76.15439624828563581, -208.4761096198365351, -353.6627254251765180 ) ) ;
#44367=CARTESIAN_POINT ( 'NONE',  ( -104.1769097210477213, -277.5132987597655756, -233.5404375194501654 ) ) ;
#44368=CARTESIAN_POINT ( 'NONE',  ( -83.08045875909370181, -284.3630566759910607, -208.7363266263961350 ) ) ;
#44369=CARTESIAN_POINT ( 'NONE',  ( -67.13259920691677962, -274.4541651701845240, -203.5259595818224057 ) ) ;
#44370=CARTESIAN_POINT ( 'NONE',  ( -60.70833197001743287, -275.1802099290781598, -197.5556040499927519 ) ) ;
#44371=CARTESIAN_POINT ( 'NONE',  ( 31.28017531377432547, -275.5531324580429100, -295.4705142078872768 ) ) ;
#44372=CARTESIAN_POINT ( 'NONE',  ( -3.409625314792581907, -296.6043879041391165, -337.2605893837646249 ) ) ;
#44373=CARTESIAN_POINT ( 'NONE',  ( -82.85093667304971632, -289.8223478022947575, -332.4731892214102800 ) ) ;
#44375=CARTESIAN_POINT ( 'NONE',  ( 29.46037816190632697, -279.1660899202661312, -234.9394982464266945 ) ) ;
#44376=CARTESIAN_POINT ( 'NONE',  ( -5.884994359699165400, -292.2876765261773926, -200.0654259477474852 ) ) ;
#44378=CARTESIAN_POINT ( 'NONE',  ( -76.00309409725149123, -288.6412777343273888, -332.5600332811768567 ) ) ;
#44379=CARTESIAN_POINT ( 'NONE',  ( 37.44861756189148139, -291.4800287172817548, -264.7567423375353997 ) ) ;
#44382=CARTESIAN_POINT ( 'NONE',  ( -109.0003189781140378, -289.8711513757135663, -284.6740238976378237 ) ) ;
#44384=CARTESIAN_POINT ( 'NONE',  ( 26.93417499958815498, -287.9403251794864218, -228.3916994810386996 ) ) ;
#44385=CARTESIAN_POINT ( 'NONE',  ( 17.40634833298267736, -296.6948066931273047, -313.9805196606274080 ) ) ;
#44386=CARTESIAN_POINT ( 'NONE',  ( 24.68905125968658254, -293.2132097090457137, -315.6049992319474882 ) ) ;
#44388=CARTESIAN_POINT ( 'NONE',  ( -5.644450957155282111, -283.9590942759782024, -339.9928827841347925 ) ) ;
#44389=CARTESIAN_POINT ( 'NONE',  ( -67.54575944813693411, -285.4778171993384603, -203.9027490203200443 ) ) ;
#44391=CARTESIAN_POINT ( 'NONE',  ( 20.42038450697154062, -277.5041895992366108, -315.8212963961043442 ) ) ;
#44392=CARTESIAN_POINT ( 'NONE',  ( 20.08265250920577927, -292.2337960397535994, -318.0506402110909221 ) ) ;
#44393=CARTESIAN_POINT ( 'NONE',  ( -65.95386005564168386, -272.4641321515136383, -202.7706244956038404 ) ) ;
#44396=CARTESIAN_POINT ( 'NONE',  ( 11.18169288377148085, -294.0680743689401879, -330.1895312541307135 ) ) ;
#44397=CARTESIAN_POINT ( 'NONE',  ( -38.67474428239044926, -287.9554958543614589, -195.9203231659482469 ) ) ;
#44398=CARTESIAN_POINT ( 'NONE',  ( -100.5039200552215135, -298.2086314536894065, -226.8406034725549034 ) ) ;
#44400=CARTESIAN_POINT ( 'NONE',  ( 25.03338392898101716, -287.6790611060463334, -232.2397124875878660 ) ) ;
#44401=CARTESIAN_POINT ( 'NONE',  ( -93.17113290953955129, -276.8886407447756710, -323.1241681779562782 ) ) ;
#44402=CARTESIAN_POINT ( 'NONE',  ( -22.10961441625129353, -295.5133499431731252, -345.7354926144147385 ) ) ;
#44403=CARTESIAN_POINT ( 'NONE',  ( 18.69446659952220102, -286.3962902350400554, -321.3731161338902211 ) ) ;
#44404=CARTESIAN_POINT ( 'NONE',  ( -11.06043674947947153, -295.0521836527204869, -342.7712458051398130 ) ) ;
#44405=CARTESIAN_POINT ( 'NONE',  ( -22.74054715544054872, -292.5774930038245429, -198.8146727979816717 ) ) ;
#44406=FACE_OUTER_BOUND ( 'NONE', #29919, .T. ) ;
#44409=CARTESIAN_POINT ( 'NONE',  ( 24.96766530141969298, -288.4837852136734000, -226.2903202452731080 ) ) ;
#44410=CARTESIAN_POINT ( 'NONE',  ( -111.2869819898779866, -287.6237833571632905, -305.9350535429201159 ) ) ;
#44412=CARTESIAN_POINT ( 'NONE',  ( -73.71010316927231543, -278.9309456273461478, -202.5918370350309772 ) ) ;
#44413=CARTESIAN_POINT ( 'NONE',  ( 21.09200081758644885, -282.9079775485607229, -223.6114546128249856 ) ) ;
#44414=CARTESIAN_POINT ( 'NONE',  ( -37.53648651393305613, -140.8450507183935372, -363.5632225393354133 ) ) ;
#44415=CARTESIAN_POINT ( 'NONE',  ( -112.9019556255240531, -283.2745553166539594, -258.6437639470820500 ) ) ;
#44416=CARTESIAN_POINT ( 'NONE',  ( 4.402289580088711851, -286.5645569975753801, -332.0572899117436236 ) ) ;
#44417=CARTESIAN_POINT ( 'NONE',  ( 4.166324136486196927, -276.4651173473556582, -206.9160032604663968 ) ) ;
#44419=CARTESIAN_POINT ( 'NONE',  ( -96.93656144539038166, -297.6341838151465709, -228.0948081563197150 ) ) ;
#44421=CARTESIAN_POINT ( 'NONE',  ( -47.88019754310063547, -293.8736607139437638, -343.1463937689038062 ) ) ;
#44422=CARTESIAN_POINT ( 'NONE',  ( -100.1704968793952730, -279.7910095877339245, -226.0231536011464186 ) ) ;
#44423=CARTESIAN_POINT ( 'NONE',  ( 19.18159363966009678, -276.2064553192546441, -316.5773227746499288 ) ) ;
#44424=CARTESIAN_POINT ( 'NONE',  ( -58.05141491136269138, -274.8704876454293640, -196.4641886117378533 ) ) ;
#44425=CARTESIAN_POINT ( 'NONE',  ( -95.92201054560364071, -276.8027795264148381, -319.8772475206681065 ) ) ;
#44427=CARTESIAN_POINT ( 'NONE',  ( -99.00777544970651434, -275.9721055732606487, -313.1379650736610643 ) ) ;
#44428=CARTESIAN_POINT ( 'NONE',  ( -96.89858719006657850, -298.6238831381976411, -222.4906312597882163 ) ) ;
#44429=CARTESIAN_POINT ( 'NONE',  ( 21.27581636871892101, -277.4090924074130839, -223.5744983911110353 ) ) ;
#44430=CARTESIAN_POINT ( 'NONE',  ( -104.5266604826868644, -260.4492150524036447, -315.3738353148558531 ) ) ;
#44431=CARTESIAN_POINT ( 'NONE',  ( -72.53443448135334393, -286.6543576803468341, -206.0374509878675156 ) ) ;
#44432=CARTESIAN_POINT ( 'NONE',  ( -111.2284843650547970, -286.0867631514931873, -288.1564007223932435 ) ) ;
#44433=CARTESIAN_POINT ( 'NONE',  ( -11.97884976289537384, -285.7397812019814864, -201.8000613284982876 ) ) ;
#44434=CARTESIAN_POINT ( 'NONE',  ( -95.09165902370692436, -276.3099652982359657, -316.3310943708975742 ) ) ;
#44435=CARTESIAN_POINT ( 'NONE',  ( -110.1449122680498647, -286.6008033708632752, -255.8505085892934119 ) ) ;
#44436=CARTESIAN_POINT ( 'NONE',  ( -107.8852716038370119, -277.3115757372997905, -249.0465155607871282 ) ) ;
#44437=CARTESIAN_POINT ( 'NONE',  ( 31.55697813618587588, -276.9658574173840293, -295.5526353879783983 ) ) ;
#44439=CARTESIAN_POINT ( 'NONE',  ( -105.4758991599336042, -273.3983116452837976, -243.8450373613339082 ) ) ;
#44440=CARTESIAN_POINT ( 'NONE',  ( 23.61295256125125519, -281.7293639233248541, -223.5561990381359578 ) ) ;
#44441=CARTESIAN_POINT ( 'NONE',  ( 39.55849578082804641, -282.0748664622238948, -272.7873851220412007 ) ) ;
#44445=CARTESIAN_POINT ( 'NONE',  ( 31.74836090790034859, -289.8162046137148309, -301.4556342819422525 ) ) ;
#44446=CARTESIAN_POINT ( 'NONE',  ( -97.94727184224944949, -289.8643234001185647, -223.6466403493475354 ) ) ;
#44447=CARTESIAN_POINT ( 'NONE',  ( -101.6140365460790207, -295.2733017846820758, -305.3134926926056210 ) ) ;
#44448=CARTESIAN_POINT ( 'NONE',  ( 1.655572977045638883, -291.9074594633247557, -204.0241312106408600 ) ) ;
#44449=CARTESIAN_POINT ( 'NONE',  ( 31.12220547957002381, -286.3950449812379588, -297.7640427143419402 ) ) ;
#44450=CARTESIAN_POINT ( 'NONE',  ( -44.07600371577404275, -287.1701884124922799, -197.2736384802797147 ) ) ;
#44451=CARTESIAN_POINT ( 'NONE',  ( 10.64812456238590066, -296.9090924074130271, -330.4860931364851808 ) ) ;
#44453=CARTESIAN_POINT ( 'NONE',  ( 32.19777683865432039, -289.9200825905789429, -298.5933697598667322 ) ) ;
#44454=CARTESIAN_POINT ( 'NONE',  ( -95.00151520645839298, -287.8870459135698070, -318.6032244064245447 ) ) ;
#44455=CARTESIAN_POINT ( 'NONE',  ( -70.31014610554780120, -284.4389455149029118, -335.7700183032857808 ) ) ;
#44456=CARTESIAN_POINT ( 'NONE',  ( -91.50904514648496502, -293.2837682530359871, -218.1724824709413326 ) ) ;
#44461=CARTESIAN_POINT ( 'NONE',  ( -35.53988309452446970, -299.9946885707460638, -194.8005259585299882 ) ) ;
#44462=CARTESIAN_POINT ( 'NONE',  ( -34.29639471325485545, -279.2885446299473529, -197.2504767746720518 ) ) ;
#44463=CARTESIAN_POINT ( 'NONE',  ( -108.0680676132336515, -282.2269498391435718, -295.4715142238394492 ) ) ;
#44464=CARTESIAN_POINT ( 'NONE',  ( 39.49491924258473574, -292.7128737016991522, -267.4529351068531469 ) ) ;
#44465=CARTESIAN_POINT ( 'NONE',  ( -81.66010341218630231, -271.6797174297837500, -211.0190601774547190 ) ) ;
#44466=CARTESIAN_POINT ( 'NONE',  ( 1.604380613884477835, -274.6074031863089431, -333.8607555102322522 ) ) ;
#44467=CARTESIAN_POINT ( 'NONE',  ( -47.35641305353401265, -299.2375501049691593, -197.5019437679379166 ) ) ;
#44469=CARTESIAN_POINT ( 'NONE',  ( -90.02586537163300306, -294.0236367781329818, -325.1907983128676847 ) ) ;
#44471=CARTESIAN_POINT ( 'NONE',  ( 35.42337767063744280, -295.1254929474005735, -281.6757419492871009 ) ) ;
#44473=CARTESIAN_POINT ( 'NONE',  ( -34.28423557078182426, -295.8155653478509635, -343.4586804439903744 ) ) ;
#44474=DIRECTION ( 'NONE',  ( 3.961265963009670520E-15, 7.202301750926674102E-15, -1.000000000000000000 ) ) ;
#44475=CARTESIAN_POINT ( 'NONE',  ( -35.16982601332965430, -284.0993750176975823, -195.0243565101894774 ) ) ;
#44476=CARTESIAN_POINT ( 'NONE',  ( -101.4673155125522044, -296.0760051309009100, -305.2452899171625518 ) ) ;
#44478=CARTESIAN_POINT ( 'NONE',  ( -81.56155594951749777, -283.6353463407463096, -333.4625159746628924 ) ) ;
#44479=CARTESIAN_POINT ( 'NONE',  ( 36.46433779166198974, -283.6793481051777235, -286.6068446237343892 ) ) ;
#44480=CARTESIAN_POINT ( 'NONE',  ( 12.39893236550466149, -288.0477611921755852, -329.1115543262658889 ) ) ;
#44481=CARTESIAN_POINT ( 'NONE',  ( 37.36665883640003472, -291.4857647391988849, -265.2150234997680514 ) ) ;
#44482=CARTESIAN_POINT ( 'NONE',  ( -114.2756510520024023, -277.9211900629985053, -268.7281209873597163 ) ) ;
#44483=CARTESIAN_POINT ( 'NONE',  ( -106.6662871844225293, -275.6237833571632905, -303.7098442033569654 ) ) ;
#44486=CARTESIAN_POINT ( 'NONE',  ( 35.84656591180441865, -286.4280063342276890, -276.5299010496783012 ) ) ;
#44487=CARTESIAN_POINT ( 'NONE',  ( -107.4543787818009690, -289.0728505083510527, -301.5675758362905299 ) ) ;
#44489=CARTESIAN_POINT ( 'NONE',  ( -88.55011191044064844, -280.7756261154848403, -213.6486426861320638 ) ) ;
#44490=CARTESIAN_POINT ( 'NONE',  ( -2.745557503210954486, -292.6171428844522211, -337.3052269194305381 ) ) ;
#44491=CARTESIAN_POINT ( 'NONE',  ( 30.35254270268198695, -281.5854002178119799, -297.7395214106401227 ) ) ;
#44492=CARTESIAN_POINT ( 'NONE',  ( -33.43271445983832280, -295.1709301181975889, -347.2749514855799475 ) ) ;
#44493=CARTESIAN_POINT ( 'NONE',  ( 30.14680484349281286, -285.1864433826016239, -236.3814786101340246 ) ) ;
#44494=CARTESIAN_POINT ( 'NONE',  ( -107.8476544276615670, -280.2189563632457521, -296.0845840191279308 ) ) ;
#44498=CARTESIAN_POINT ( 'NONE',  ( -108.6533021207399941, -295.8503018677580485, -286.2558926937859951 ) ) ;
#44500=CARTESIAN_POINT ( 'NONE',  ( -69.85430415644619018, -277.1237833571632905, -202.7746430608542312 ) ) ;
#44501=CARTESIAN_POINT ( 'NONE',  ( -68.76864842908555886, -272.8466325309435092, -200.2289550064433001 ) ) ;
#44502=CARTESIAN_POINT ( 'NONE',  ( -105.1138348963155096, -290.0207650408347035, -297.6249682552959825 ) ) ;
#44503=CARTESIAN_POINT ( 'NONE',  ( -108.6483298486302971, -280.3161605161693046, -251.7084807321710116 ) ) ;
#44504=CARTESIAN_POINT ( 'NONE',  ( -3.758639256968665521, -276.1029865031083546, -204.6307367993258310 ) ) ;
#44505=CARTESIAN_POINT ( 'NONE',  ( -8.324456075631273322, -284.2787723166438809, -340.8758594970555578 ) ) ;
#44506=CARTESIAN_POINT ( 'NONE',  ( 34.96087503310251066, -280.1813885121293310, -257.7330488293075632 ) ) ;
#44507=CARTESIAN_POINT ( 'NONE',  ( -5.402396971767837286, -278.6321329417295942, -338.2345440956249263 ) ) ;
#44509=CARTESIAN_POINT ( 'NONE',  ( -44.04064290410936167, -273.8031295698629606, -193.5997647266876811 ) ) ;
#44510=CARTESIAN_POINT ( 'NONE',  ( -84.76485457830875703, -293.3126168828366644, -212.9820397666364897 ) ) ;
#44514=CARTESIAN_POINT ( 'NONE',  ( -8.874483681549044434, -292.8234407389844591, -340.6300956179244963 ) ) ;
#44515=CARTESIAN_POINT ( 'NONE',  ( -34.03162291124731809, -273.6025578906466080, -197.3745998397894823 ) ) ;
#44518=CARTESIAN_POINT ( 'NONE',  ( -40.62216451258591832, -293.5317462503446677, -194.1119325345804043 ) ) ;
#44519=CARTESIAN_POINT ( 'NONE',  ( -95.99890600148557951, -281.6948066931273615, -223.6242672951989618 ) ) ;
#44520=CARTESIAN_POINT ( 'NONE',  ( -14.00211361193672488, -293.5533089795849833, -197.3446760585814559 ) ) ;
#44521=CARTESIAN_POINT ( 'NONE',  ( 31.64215255283919248, -289.1710774764609937, -241.2226099136157984 ) ) ;
#44522=CARTESIAN_POINT ( 'NONE',  ( 37.47637329432973985, -273.5325373212593831, -268.8497236634133287 ) ) ;
#44523=CARTESIAN_POINT ( 'NONE',  ( 8.485773122936732804, -278.3396286921513365, -329.0881921755071744 ) ) ;
#44524=CARTESIAN_POINT ( 'NONE',  ( -15.18712578377499867, -292.8430217246077518, -341.4821248836370273 ) ) ;
#44525=CARTESIAN_POINT ( 'NONE',  ( -97.60846626097666956, -281.0348212588008323, -224.4245933156176989 ) ) ;
#44527=CARTESIAN_POINT ( 'NONE',  ( -99.05117690618099857, -283.6784212986337366, -309.4945871985907502 ) ) ;
#44528=CARTESIAN_POINT ( 'NONE',  ( -99.18677729593699155, -280.2367619352089605, -224.9883271627897159 ) ) ;
#44529=CARTESIAN_POINT ( 'NONE',  ( -21.82150746302388455, -281.6524179623428381, -345.3753322163662460 ) ) ;
#44531=CARTESIAN_POINT ( 'NONE',  ( -4.085903519213418988, -277.5655622886697529, -339.5627995235928438 ) ) ;
#44532=CARTESIAN_POINT ( 'NONE',  ( 33.54740286788948112, -277.4353878861709859, -298.7426974221996261 ) ) ;
#44533=CARTESIAN_POINT ( 'NONE',  ( 7.450504543161046378, -284.9090924074130839, -326.4764044574609443 ) ) ;
#44536=CARTESIAN_POINT ( 'NONE',  ( -95.21197722736944513, -275.2080839337588145, -222.8957426162362196 ) ) ;
#44537=CARTESIAN_POINT ( 'NONE',  ( -97.02097982478332483, -292.2251515782290880, -227.7004791358921523 ) ) ;
#44538=CARTESIAN_POINT ( 'NONE',  ( -111.5997290360169956, -276.6765306270784777, -262.2784132876439003 ) ) ;
#44539=CARTESIAN_POINT ( 'NONE',  ( -48.69515949728628357, -290.9548249376470608, -345.5480509916260985 ) ) ;
#44540=CARTESIAN_POINT ( 'NONE',  ( -62.82850568139382119, -291.0599634610347266, -201.8460436494954138 ) ) ;
#44541=CARTESIAN_POINT ( 'NONE',  ( -14.97613394031227685, -288.2777900849700359, -344.0327749128680921 ) ) ;
#44543=CARTESIAN_POINT ( 'NONE',  ( -98.20353022599101678, -282.3762547052830882, -312.1908215390862438 ) ) ;
#44544=CARTESIAN_POINT ( 'NONE',  ( -108.9495300949364918, -292.6668875430676735, -250.7860274442684840 ) ) ;
#44545=CARTESIAN_POINT ( 'NONE',  ( -60.17525078554039908, -284.2305803015421475, -200.2944588943720134 ) ) ;
#44546=CARTESIAN_POINT ( 'NONE',  ( 25.54968415209746269, -282.3462423541583348, -232.2373147414432424 ) ) ;
#44547=CARTESIAN_POINT ( 'NONE',  ( -74.30347451398851888, -290.4724224527875549, -337.6564888963608837 ) ) ;
#44548=CARTESIAN_POINT ( 'NONE',  ( -41.06058262325050379, -280.4964356004866772, -197.3942874719873259 ) ) ;
#44549=CARTESIAN_POINT ( 'NONE',  ( -27.88282330290596533, -290.9644974789804905, -194.2910214177152284 ) ) ;
#44550=CARTESIAN_POINT ( 'NONE',  ( 39.54105710971416698, -288.3697402850789331, -271.5385890454601849 ) ) ;
#44551=CARTESIAN_POINT ( 'NONE',  ( 3.153082315061669139, -289.0163810657550130, -335.8430311126187462 ) ) ;
#44552=CARTESIAN_POINT ( 'NONE',  ( -5.800571593454897368, -286.6454022889337239, -204.5130177428107174 ) ) ;
#44555=CARTESIAN_POINT ( 'NONE',  ( -5.007819722550730823, -296.4914400188387162, -338.8941561392257995 ) ) ;
#44556=CARTESIAN_POINT ( 'NONE',  ( -88.28959555612692611, -294.4327322491347445, -327.5076521907544134 ) ) ;
#44557=CARTESIAN_POINT ( 'NONE',  ( -18.96945557316667674, -275.8685172346219474, -341.2544821108269275 ) ) ;
#44558=CARTESIAN_POINT ( 'NONE',  ( -102.2259323693968014, -296.4424229146545144, -229.0894667808400982 ) ) ;
#44559=CARTESIAN_POINT ( 'NONE',  ( 23.49451730750386247, -292.6063665550602195, -312.0395319126256481 ) ) ;
#44560=CARTESIAN_POINT ( 'NONE',  ( -109.4594346524990698, -295.0085612084535569, -253.7176092238774174 ) ) ;
#44561=CARTESIAN_POINT ( 'NONE',  ( 34.87109307281083659, -294.5840231894339922, -257.1595545445645143 ) ) ;
#44562=CARTESIAN_POINT ( 'NONE',  ( 29.77856839255682786, -295.0267540612816219, -299.8415458359543209 ) ) ;
#44564=CARTESIAN_POINT ( 'NONE',  ( -37.70627606878536398, -293.0565156026447085, -345.5396714588636655 ) ) ;
#44565=CARTESIAN_POINT ( 'NONE',  ( 82.12347693879148380, -301.5478687382300222, -195.3203844934047311 ) ) ;
#44566=CARTESIAN_POINT ( 'NONE',  ( -66.41143275288175118, -290.3835155073352325, -337.6340440660973741 ) ) ;
#44567=CARTESIAN_POINT ( 'NONE',  ( -73.30912404235306212, -295.8766123599677940, -333.9097757478731978 ) ) ;
#44568=CARTESIAN_POINT ( 'NONE',  ( -108.1817001848615405, -280.1986913336840530, -296.2060549065487294 ) ) ;
#44569=CARTESIAN_POINT ( 'NONE',  ( -68.45652880106044336, -278.3366787867803396, -200.4528655925653595 ) ) ;
#44571=CARTESIAN_POINT ( 'NONE',  ( -109.0685185281854643, -272.2540321755280388, -242.4913780628532152 ) ) ;
#44572=CARTESIAN_POINT ( 'NONE',  ( 23.30051269408180659, -279.0406177156627336, -227.1889484361012705 ) ) ;
#44573=CARTESIAN_POINT ( 'NONE',  ( -77.05797299808246237, -277.9296433904203241, -205.2688336345278799 ) ) ;
#44574=CARTESIAN_POINT ( 'NONE',  ( -104.5252511496972545, -276.9975555567187939, -236.5347552008784362 ) ) ;
#44576=CARTESIAN_POINT ( 'NONE',  ( -102.5441727504278617, -271.5887871775647113, -236.1331745616857063 ) ) ;
#44577=CARTESIAN_POINT ( 'NONE',  ( -112.1889503641107950, -274.6232853802811746, -264.8338837743303316 ) ) ;
#44579=CARTESIAN_POINT ( 'NONE',  ( -112.1831259452708736, -288.4544794835377388, -279.5775346463707933 ) ) ;
#44580=CARTESIAN_POINT ( 'NONE',  ( -74.42731838132610278, -289.5313224861060348, -337.8569607667662353 ) ) ;
#44581=CARTESIAN_POINT ( 'NONE',  ( -2.182146302530975746, -276.5166566984440806, -203.9244247787239601 ) ) ;
#44582=CARTESIAN_POINT ( 'NONE',  ( -35.05284281979317029, -296.0807104606674329, -195.5285584408348711 ) ) ;
#44583=CARTESIAN_POINT ( 'NONE',  ( -109.8215417628479287, -284.0718311411624200, -244.8497209834165460 ) ) ;
#44585=CARTESIAN_POINT ( 'NONE',  ( -4.537303454627476640, -280.6198067724292287, -337.8204163905774067 ) ) ;
#44587=CARTESIAN_POINT ( 'NONE',  ( -33.47223843021657785, -290.8968293585060110, -197.0535528786665225 ) ) ;
#44588=CARTESIAN_POINT ( 'NONE',  ( -41.36660575354350300, -284.1405522321418857, -196.2223962516110589 ) ) ;
#44590=CARTESIAN_POINT ( 'NONE',  ( 128.9960186029002500, -299.5541904835127980, -201.1130027942871266 ) ) ;
#44591=CARTESIAN_POINT ( 'NONE',  ( -27.82807646614444863, -290.1726618137871014, -195.9148144460450283 ) ) ;
#44592=CARTESIAN_POINT ( 'NONE',  ( -95.89544874472140634, -279.5271080104831753, -315.2821480264194633 ) ) ;
#44593=CARTESIAN_POINT ( 'NONE',  ( 4.342564639707441998, -283.7089005723038326, -334.6922459569185548 ) ) ;
#44594=CARTESIAN_POINT ( 'NONE',  ( -54.97342816398631982, -271.9070030809024843, -196.8870656809470461 ) ) ;
#44595=CARTESIAN_POINT ( 'NONE',  ( -108.9289666493128976, -284.7406883148457837, -256.0690477330068688 ) ) ;
#44597=CARTESIAN_POINT ( 'NONE',  ( -11.02651898563433441, -278.1275328455262752, -339.0843757538093541 ) ) ;
#44598=CARTESIAN_POINT ( 'NONE',  ( -64.38333566952888987, -278.2170181170437218, -338.3954395343232591 ) ) ;
#44599=CARTESIAN_POINT ( 'NONE',  ( -94.72325778133917140, -285.8844174726269785, -318.6754674865924812 ) ) ;
#44603=CARTESIAN_POINT ( 'NONE',  ( -112.6000473950164888, -296.5898526349620283, -254.0152002827317688 ) ) ;
#44604=CARTESIAN_POINT ( 'NONE',  ( -1.416422438511701021, -288.5104897743728998, -204.8720907206462414 ) ) ;
#44606=CARTESIAN_POINT ( 'NONE',  ( -72.08107566293803359, -292.9809262143061233, -342.4248175857292154 ) ) ;
#44607=CARTESIAN_POINT ( 'NONE',  ( -107.1320942456446090, -277.8819512006079435, -238.4403332413932901 ) ) ;
#44608=CARTESIAN_POINT ( 'NONE',  ( -81.45054519529385573, -289.8629449931410136, -208.2253778607089032 ) ) ;
#44609=CARTESIAN_POINT ( 'NONE',  ( -79.72370072472189406, -286.9881181221589941, -210.0118627776461722 ) ) ;
#44611=CARTESIAN_POINT ( 'NONE',  ( -68.97646978270985585, -281.3904523356027880, -203.4491208114842777 ) ) ;
#44612=CARTESIAN_POINT ( 'NONE',  ( 35.28327770688060383, -288.6743423350946500, -246.4387367549829548 ) ) ;
#44613=CARTESIAN_POINT ( 'NONE',  ( 37.56466911442159784, -283.6004216151127935, -274.1076487702263194 ) ) ;
#44614=CARTESIAN_POINT ( 'NONE',  ( -39.96082666270670103, -277.2508535597563650, -347.3296270181057821 ) ) ;
#44615=CARTESIAN_POINT ( 'NONE',  ( -95.72232120735915828, -295.2146963515584162, -223.8471427734565680 ) ) ;
#44616=CARTESIAN_POINT ( 'NONE',  ( -109.6054548109871263, -278.7232482755541128, -243.6186671819040441 ) ) ;
#44617=CARTESIAN_POINT ( 'NONE',  ( -13.69402298196853529, -276.2228071967882670, -199.9931363106979347 ) ) ;
#44621=CARTESIAN_POINT ( 'NONE',  ( -106.6662871844225293, -287.4805209788416391, -237.0123917617630980 ) ) ;
#44622=CARTESIAN_POINT ( 'NONE',  ( -49.53425585000079678, -272.1387402999603751, -195.3059184839057139 ) ) ;
#44624=CARTESIAN_POINT ( 'NONE',  ( -87.56838295377406212, -278.8359714518171586, -217.2321004917276923 ) ) ;
#44625=CARTESIAN_POINT ( 'NONE',  ( 14.62513591415104663, -277.5453004359696934, -326.7134886409957630 ) ) ;
#44626=CARTESIAN_POINT ( 'NONE',  ( -21.78541642493446773, -281.9161992435768411, -345.5330691986537772 ) ) ;
#44627=CARTESIAN_POINT ( 'NONE',  ( 20.31681896614901817, -289.9593618248425173, -316.7666046462033478 ) ) ;
#44628=CARTESIAN_POINT ( 'NONE',  ( -93.16883987994312122, -298.7885027996163672, -218.2644281607912546 ) ) ;
#44629=CARTESIAN_POINT ( 'NONE',  ( -106.1633422266400828, -298.1914197729561238, -236.7219994400396672 ) ) ;
#44630=CARTESIAN_POINT ( 'NONE',  ( 37.25392819670436495, -295.6290118142692336, -276.3210390607483760 ) ) ;
#44631=CARTESIAN_POINT ( 'NONE',  ( 18.44613789808553861, -278.8559449414447613, -220.4838129597063698 ) ) ;
#44632=CARTESIAN_POINT ( 'NONE',  ( -65.15884029580085723, -271.7069913710247988, -201.0793533605327355 ) ) ;
#44633=CARTESIAN_POINT ( 'NONE',  ( -111.4364158034859429, -285.9267762441473337, -288.2043090941172068 ) ) ;
#44634=CARTESIAN_POINT ( 'NONE',  ( -50.82173890067777933, -288.1486111645336337, -342.4721225434952885 ) ) ;
#44635=CARTESIAN_POINT ( 'NONE',  ( 203.4894716936504722, 292.6718879101889570, -83.16901316872426264 ) ) ;
#44636=ORIENTED_EDGE ( 'NONE', *, *, #7316, .F. ) ;
#44637=CARTESIAN_POINT ( 'NONE',  ( 35.81596198814759191, -286.4063980440811861, -292.4646931912116656 ) ) ;
#44638=CARTESIAN_POINT ( 'NONE',  ( -8.213959618484716785, -288.3267408992413721, -337.3753253256066955 ) ) ;
#44640=CARTESIAN_POINT ( 'NONE',  ( -97.34717193201876739, -286.2737686607163141, -222.6030206056668987 ) ) ;
#44641=CARTESIAN_POINT ( 'NONE',  ( -37.80563493136995135, -277.3913669075303119, -343.3932448444861052 ) ) ;
#44643=CARTESIAN_POINT ( 'NONE',  ( 23.73741687090086216, -291.8517634764929767, -223.9624184666445217 ) ) ;
#44644=CARTESIAN_POINT ( 'NONE',  ( 29.67713935713489448, -282.6946486322358396, -308.1762652143417540 ) ) ;
#44645=CARTESIAN_POINT ( 'NONE',  ( 31.77270039375430954, -283.4915360243597320, -302.8261636814642088 ) ) ;
#44646=CARTESIAN_POINT ( 'NONE',  ( -81.54594247968130105, -283.9685738634240124, -333.4476209434370162 ) ) ;
#44647=CARTESIAN_POINT ( 'NONE',  ( -27.55974336206074327, -280.5129850451773450, -197.9469330038109831 ) ) ;
#44648=CARTESIAN_POINT ( 'NONE',  ( 26.53690525259170840, -296.4086741954485547, -200.3901485728259502 ) ) ;
#44649=CARTESIAN_POINT ( 'NONE',  ( 180.4107272569747522, 254.1056192471400834, -166.8072156021353862 ) ) ;
#44651=CARTESIAN_POINT ( 'NONE',  ( -36.41863139110428449, -279.0407500586431979, -345.2015424416197789 ) ) ;
#44652=CARTESIAN_POINT ( 'NONE',  ( 44.12337886667094722, 12.84550829123691607, -331.4150732913272464 ) ) ;
#44653=CARTESIAN_POINT ( 'NONE',  ( 172.1664621943805855, 241.6173149327171927, -177.3709744135503570 ) ) ;
#44654=CARTESIAN_POINT ( 'NONE',  ( -109.8362118316587441, -296.0296523786192324, -260.5748814699558125 ) ) ;
#44655=CARTESIAN_POINT ( 'NONE',  ( 37.39872793009974572, -293.2890167128820167, -288.6753417241641841 ) ) ;
#44656=CARTESIAN_POINT ( 'NONE',  ( -76.03803979523620171, -208.5652239327323230, -353.7424279183983344 ) ) ;
#44657=CARTESIAN_POINT ( 'NONE',  ( -97.75683960899084468, -295.7565143839406687, -223.5573490943200170 ) ) ;
#44658=CARTESIAN_POINT ( 'NONE',  ( -87.28560909400981416, -288.1617947099340995, -324.7632003716275335 ) ) ;
#44659=CARTESIAN_POINT ( 'NONE',  ( -36.96589763307245136, -296.9077808332467612, -344.6080054043234782 ) ) ;
#44660=CARTESIAN_POINT ( 'NONE',  ( 35.94505693686367209, -288.9478502166791714, -276.5060089043064977 ) ) ;
#44662=CARTESIAN_POINT ( 'NONE',  ( -56.00145377709480954, -296.2280420907616190, -344.8234158657631383 ) ) ;
#44663=CARTESIAN_POINT ( 'NONE',  ( -10.73339725628381913, -286.9010971248844726, -202.3035759172179269 ) ) ;
#44664=CARTESIAN_POINT ( 'NONE',  ( 19.04079931267920500, -297.5382118137887346, -193.7694208783678960 ) ) ;
#44665=CARTESIAN_POINT ( 'NONE',  ( -25.05735014571818908, -293.0078349272711762, -194.5109131998279679 ) ) ;
#44666=CARTESIAN_POINT ( 'NONE',  ( 21.32479549574819799, -294.7160000565395421, -320.1383135106926829 ) ) ;
#44667=CARTESIAN_POINT ( 'NONE',  ( -90.76063324359087403, -291.4343998394230653, -220.5890667451404852 ) ) ;
#44670=CARTESIAN_POINT ( 'NONE',  ( -24.43018444405199929, -276.1357367808887489, -195.8592807407198677 ) ) ;
#44671=CARTESIAN_POINT ( 'NONE',  ( 33.80971135660507798, -274.7106289550790166, -298.8851311009365759 ) ) ;
#44673=CARTESIAN_POINT ( 'NONE',  ( -74.07299186125582935, -277.0344159499891248, -337.9803917655460737 ) ) ;
#44674=CARTESIAN_POINT ( 'NONE',  ( -37.12834905313825828, -296.5347552425564572, -196.6649599176964784 ) ) ;
#44675=CARTESIAN_POINT ( 'NONE',  ( -67.32288110887056121, -275.5891577717744667, -338.2727831776886092 ) ) ;
#44676=CARTESIAN_POINT ( 'NONE',  ( -108.2425790858671348, -273.8791828732166209, -251.5305680901520589 ) ) ;
#44677=CARTESIAN_POINT ( 'NONE',  ( -40.79800506375547542, -274.9490062376215178, -197.1575673354057869 ) ) ;
#44678=CARTESIAN_POINT ( 'NONE',  ( -78.31426933644966937, -275.2691208377483463, -206.3671918259205711 ) ) ;
#44679=CARTESIAN_POINT ( 'NONE',  ( -57.65349535606151932, -271.8114165114203615, -197.7407897154428440 ) ) ;
#44680=CARTESIAN_POINT ( 'NONE',  ( -108.6895465585165397, -296.9938770632317642, -286.2789532096331868 ) ) ;
#44681=CARTESIAN_POINT ( 'NONE',  ( -5.301236082398643745, -293.1967711233344289, -336.6229329529934375 ) ) ;
#44683=CARTESIAN_POINT ( 'NONE',  ( 23.47326059264479881, -276.6745026864238639, -317.5106893298946034 ) ) ;
#44684=CARTESIAN_POINT ( 'NONE',  ( -8.972789955045374910, -274.6003677338711100, -203.0449969625420010 ) ) ;
#44686=CARTESIAN_POINT ( 'NONE',  ( -68.28584703499974751, -284.3389852862416660, -200.3771416406644619 ) ) ;
#44687=CARTESIAN_POINT ( 'NONE',  ( -110.4961289190214160, -298.7736498809231307, -253.0851815561672709 ) ) ;
#44689=CARTESIAN_POINT ( 'NONE',  ( -6.940097155144616892, -285.6587834874952136, -203.8015540110765755 ) ) ;
#44690=CARTESIAN_POINT ( 'NONE',  ( -85.78519100076424309, -275.9731597293535401, -326.3861723131170720 ) ) ;
#44691=CARTESIAN_POINT ( 'NONE',  ( -110.7575939558557252, -277.0516825539775709, -276.1069616884851143 ) ) ;
#44692=CARTESIAN_POINT ( 'NONE',  ( 21.21648027691207261, -284.1969157558150414, -317.2421113133214590 ) ) ;
#44693=CARTESIAN_POINT ( 'NONE',  ( -1.542295531487216209, -275.7430442908468535, -206.2722937548323046 ) ) ;
#44695=CARTESIAN_POINT ( 'NONE',  ( 22.00497724944198552, -274.5995621614944753, -318.1772756555577075 ) ) ;
#44696=CARTESIAN_POINT ( 'NONE',  ( -56.12377700401275860, -281.8110800841286618, -197.5251300938368502 ) ) ;
#44698=CARTESIAN_POINT ( 'NONE',  ( -54.65878368267649989, -287.7514365363581419, -196.8122715449479472 ) ) ;
#44700=CARTESIAN_POINT ( 'NONE',  ( -68.09640297299399947, -289.6482022707571673, -201.9429564497393130 ) ) ;
#44702=CARTESIAN_POINT ( 'NONE',  ( -85.62160426803460211, -272.0527504544953104, -214.8830665554402515 ) ) ;
#44703=CARTESIAN_POINT ( 'NONE',  ( -60.62426123480083362, -289.8866211824146149, -199.8175581276832418 ) ) ;
#44704=CARTESIAN_POINT ( 'NONE',  ( -101.2450674239233592, -254.4445186991787295, -323.9438275447045612 ) ) ;
#44706=CARTESIAN_POINT ( 'NONE',  ( 31.05727500542148789, -286.4720547611850634, -304.3075498103050904 ) ) ;
#44707=CARTESIAN_POINT ( 'NONE',  ( -32.06842260366386910, -284.5846534396746392, -343.9724823211214471 ) ) ;
#44708=CARTESIAN_POINT ( 'NONE',  ( -70.60218817851117024, -283.8594481473888322, -202.0404479599195042 ) ) ;
#44709=CARTESIAN_POINT ( 'NONE',  ( -69.01760083171541282, -291.6236601841486618, -204.5777373949150046 ) ) ;
#44710=CARTESIAN_POINT ( 'NONE',  ( 35.28801081261830319, -283.1324308091676585, -282.2059483491906917 ) ) ;
#44711=CARTESIAN_POINT ( 'NONE',  ( 33.11771182293239235, -282.6147824746102515, -290.0606863735500269 ) ) ;
#44712=CARTESIAN_POINT ( 'NONE',  ( -31.91940922578854511, -290.9640783308745426, -345.5724175824318536 ) ) ;
#44713=CARTESIAN_POINT ( 'NONE',  ( -23.36195680614620684, -298.3893324513517200, -193.3607339042446540 ) ) ;
#44715=CARTESIAN_POINT ( 'NONE',  ( -18.11478860929830148, -286.8860449579979672, -343.4339588246510289 ) ) ;
#44716=CARTESIAN_POINT ( 'NONE',  ( 39.63086186175308256, -275.5264464585653741, -268.3057103049698640 ) ) ;
#44717=CARTESIAN_POINT ( 'NONE',  ( -60.79924813879813428, -293.7263106862739050, -199.4436958951495740 ) ) ;
#44719=CARTESIAN_POINT ( 'NONE',  ( -20.19161114001083490, -297.3376638359846424, -345.3538533559490702 ) ) ;
#44720=CARTESIAN_POINT ( 'NONE',  ( -23.99223936933285017, -281.5628720852006381, -342.6316885778049368 ) ) ;
#44721=CARTESIAN_POINT ( 'NONE',  ( -61.83329689734288337, -275.3694319706043530, -341.4807822853480275 ) ) ;
#44723=CARTESIAN_POINT ( 'NONE',  ( -113.5665141736607637, -294.9259093960350242, -272.4275516044332903 ) ) ;
#44724=CARTESIAN_POINT ( 'NONE',  ( 35.74498614642443783, -274.8810675183170247, -268.8681487109377031 ) ) ;
#44725=CARTESIAN_POINT ( 'NONE',  ( -57.86643658045814931, -293.3024744560507884, -199.5303163994831550 ) ) ;
#44726=CARTESIAN_POINT ( 'NONE',  ( 8.988454232498714447, -293.6470273010241954, -213.5774049988777392 ) ) ;
#44727=CARTESIAN_POINT ( 'NONE',  ( -109.6597734657279517, -286.5179925544603634, -254.5516204331351275 ) ) ;
#44728=CARTESIAN_POINT ( 'NONE',  ( 38.85213999318408185, -294.9049098300262131, -264.6074218465794274 ) ) ;
#44729=CARTESIAN_POINT ( 'NONE',  ( 17.22166499399533635, -295.6089827009751616, -324.0661191648778185 ) ) ;
#44730=CARTESIAN_POINT ( 'NONE',  ( -66.05509232820192267, -295.2720244408669714, -337.4769962296836070 ) ) ;
#44731=CARTESIAN_POINT ( 'NONE',  ( -88.06372293221394898, -291.7615039317842047, -325.6789649307979175 ) ) ;
#44732=CARTESIAN_POINT ( 'NONE',  ( -55.70012464209018077, -283.4488524062487045, -345.1405821010450836 ) ) ;
#44733=CARTESIAN_POINT ( 'NONE',  ( -36.88264727789704267, -296.1377079819332039, -194.8012588250561521 ) ) ;
#44734=CARTESIAN_POINT ( 'NONE',  ( -104.4180584499296458, -283.8935991299841817, -308.2813115394941974 ) ) ;
#44735=CARTESIAN_POINT ( 'NONE',  ( -94.85763323616953357, -279.8721596840393318, -317.9601673568814704 ) ) ;
#44736=CARTESIAN_POINT ( 'NONE',  ( -110.6236579043854391, -283.4118556721556956, -265.4232834957563796 ) ) ;
#44737=CARTESIAN_POINT ( 'NONE',  ( 25.47688555729405380, -284.9993870828847093, -229.3876394770667275 ) ) ;
#44738=CARTESIAN_POINT ( 'NONE',  ( -106.2851385975139635, -277.1013322941293495, -238.8166198569192886 ) ) ;
#44740=CARTESIAN_POINT ( 'NONE',  ( -107.4527420557531485, -283.7875800675814730, -290.9589078047928865 ) ) ;
#44741=CARTESIAN_POINT ( 'NONE',  ( 29.42339311803416990, -283.2482220161219857, -308.0249686546339944 ) ) ;
#44742=CARTESIAN_POINT ( 'NONE',  ( -1.919984878073659917, -287.6533100300147794, -338.4648792764691621 ) ) ;
#44743=CARTESIAN_POINT ( 'NONE',  ( -79.76372037430267881, -279.2150229643513626, -333.7240142589708398 ) ) ;
#44744=CARTESIAN_POINT ( 'NONE',  ( -59.50603922779158950, -278.6485014039391217, -343.5870720149753765 ) ) ;
#44745=CARTESIAN_POINT ( 'NONE',  ( -70.93977880302659855, -279.4292542214962509, -205.5383189467578688 ) ) ;
#44746=CARTESIAN_POINT ( 'NONE',  ( -21.61145548622377177, -276.2347099145011384, -197.3925891287979653 ) ) ;
#44747=CARTESIAN_POINT ( 'NONE',  ( 36.36968895583773786, -293.8336313973234724, -292.8045129553890433 ) ) ;
#44748=CARTESIAN_POINT ( 'NONE',  ( 37.51496625655154560, -285.5252883449841192, -268.2864241490587460 ) ) ;
#44750=CARTESIAN_POINT ( 'NONE',  ( -64.12688193265761072, -293.3087435754818557, -198.9683332250135379 ) ) ;
#44751=CARTESIAN_POINT ( 'NONE',  ( 29.76753150895131128, -292.8677587994326927, -299.8666615598075964 ) ) ;
#44752=CARTESIAN_POINT ( 'NONE',  ( 32.76928783810420498, -293.4892996287213123, -290.8152853006679379 ) ) ;
#44753=CARTESIAN_POINT ( 'NONE',  ( -94.49017891993483431, -292.3283144061011853, -219.2187296741897740 ) ) ;
#44754=CARTESIAN_POINT ( 'NONE',  ( 23.76318053072366610, -281.6469269062584431, -230.1439659249684269 ) ) ;
#44756=CARTESIAN_POINT ( 'NONE',  ( -93.96358585662680696, -272.3182801167610592, -218.5075328834848847 ) ) ;
#44757=CARTESIAN_POINT ( 'NONE',  ( 28.60685175407669689, -287.6859457337085928, -230.7097191566026595 ) ) ;
#44758=CARTESIAN_POINT ( 'NONE',  ( 21.54798034489373038, -280.3416052439997657, -318.0503424261314649 ) ) ;
#44759=CARTESIAN_POINT ( 'NONE',  ( 23.27343695480106689, -288.5200472869787518, -317.8328387135502453 ) ) ;
#44760=CARTESIAN_POINT ( 'NONE',  ( -71.19179091716839025, -285.9255657695690616, -205.6598132011637574 ) ) ;
#44761=FACE_OUTER_BOUND ( 'NONE', #88514, .T. ) ;
#44762=CARTESIAN_POINT ( 'NONE',  ( -14.33830847277128662, -91.16400973458658541, -357.8324979133209354 ) ) ;
#44763=CARTESIAN_POINT ( 'NONE',  ( -82.89404955411457365, -218.6374574953077570, -348.8632550632670473 ) ) ;
#44764=CARTESIAN_POINT ( 'NONE',  ( -105.4217893198336782, -277.3918462768014592, -297.1511008538128635 ) ) ;
#44765=CARTESIAN_POINT ( 'NONE',  ( -110.5895536243074986, -277.4331145171180424, -273.3574542330976556 ) ) ;
#44766=CARTESIAN_POINT ( 'NONE',  ( -30.48509448647785547, -297.6434982183235434, -193.4232108530147229 ) ) ;
#44767=CARTESIAN_POINT ( 'NONE',  ( -96.95894580772622362, -247.6687050397709129, -332.0224721523202902 ) ) ;
#44768=CARTESIAN_POINT ( 'NONE',  ( -67.52953661069818736, -276.1248168577565139, -340.6604266715875724 ) ) ;
#44769=CARTESIAN_POINT ( 'NONE',  ( -78.90372080204622307, -297.3643163006117334, -333.9737932112203680 ) ) ;
#44770=CARTESIAN_POINT ( 'NONE',  ( -93.49115227342161916, -291.7073450886715591, -223.5951683252780526 ) ) ;
#44771=CARTESIAN_POINT ( 'NONE',  ( -48.95569808031642367, -298.7107656020162381, -194.3518271525058765 ) ) ;
#44772=CARTESIAN_POINT ( 'NONE',  ( -66.54026285516115991, -288.1274541424928088, -337.8594634240878918 ) ) ;
#44773=CARTESIAN_POINT ( 'NONE',  ( -14.83877591472487012, -298.8191636796547073, -193.4208306832735502 ) ) ;
#44774=CARTESIAN_POINT ( 'NONE',  ( -108.5914054341570392, -296.5092223847959758, -286.2507214494972914 ) ) ;
#44777=CARTESIAN_POINT ( 'NONE',  ( -111.3129590246118426, -280.6695308242854594, -254.8854119829896945 ) ) ;
#44778=CARTESIAN_POINT ( 'NONE',  ( -99.42960280185914712, -279.0946903869648281, -309.4343484115653382 ) ) ;
#44779=CARTESIAN_POINT ( 'NONE',  ( -88.51295616188255622, -279.5183081714269520, -326.5347467389992744 ) ) ;
#44780=CARTESIAN_POINT ( 'NONE',  ( -87.79400934037354887, -271.8119228288654767, -216.5765389216107621 ) ) ;
#44783=CARTESIAN_POINT ( 'NONE',  ( -4.349468131463234855, -280.6662493064595765, -205.2280084688505326 ) ) ;
#44784=CARTESIAN_POINT ( 'NONE',  ( 21.72016852956733501, -275.6924834627180871, -221.2097752563675215 ) ) ;
#44785=CARTESIAN_POINT ( 'NONE',  ( 18.40806390262041248, -278.2515910834043211, -320.5497030182786489 ) ) ;
#44786=CARTESIAN_POINT ( 'NONE',  ( -98.34406267571065996, -276.5091596740006707, -316.3969231582526618 ) ) ;
#44789=CARTESIAN_POINT ( 'NONE',  ( -3.606082695485143930, -284.5891196346562992, -337.7573191692628143 ) ) ;
#44790=CARTESIAN_POINT ( 'NONE',  ( -105.8582764708482244, -290.0925123653496485, -244.5643403522202846 ) ) ;
#44791=CARTESIAN_POINT ( 'NONE',  ( -40.80356843434887537, -285.3584038721391494, -193.4888905030086050 ) ) ;
#44792=CARTESIAN_POINT ( 'NONE',  ( -85.53839468222153641, -281.9694747034328657, -326.5309732887333780 ) ) ;
#44793=CARTESIAN_POINT ( 'NONE',  ( -96.40543317635200538, -282.5161207291093319, -314.2570216278494399 ) ) ;
#44794=CARTESIAN_POINT ( 'NONE',  ( -1.787096532268313887, -281.7395368591172655, -206.1505217501277514 ) ) ;
#44795=CARTESIAN_POINT ( 'NONE',  ( 64.47034096727303165, 48.08436259181641503, -318.7852478153986908 ) ) ;
#44796=CARTESIAN_POINT ( 'NONE',  ( -81.11879237899330519, -282.0354755576044568, -332.7952388372868882 ) ) ;
#44797=CARTESIAN_POINT ( 'NONE',  ( 27.72748973062332212, -295.0547921759773544, -233.0649897977404805 ) ) ;
#44798=CARTESIAN_POINT ( 'NONE',  ( -62.60970155663485315, -287.7242411621383553, -199.5687700240574145 ) ) ;
#44802=CARTESIAN_POINT ( 'NONE',  ( -6.497557358764993296, -294.3741731780079931, -201.3691821394449164 ) ) ;
#44803=CARTESIAN_POINT ( 'NONE',  ( 27.08083609230942912, -274.0659118144562285, -308.7634287702098845 ) ) ;
#44804=CARTESIAN_POINT ( 'NONE',  ( 25.71332827411659849, -287.3318785423260238, -314.3639847695816343 ) ) ;
#44805=CARTESIAN_POINT ( 'NONE',  ( -32.08013147951756139, -290.5194624245420982, -196.7361571637703719 ) ) ;
#44807=CARTESIAN_POINT ( 'NONE',  ( -108.0885160136129599, -277.4988490640187706, -250.4114605798086188 ) ) ;
#44808=CARTESIAN_POINT ( 'NONE',  ( -102.2838809488369662, -295.1751045264184086, -234.3975443534600345 ) ) ;
#44809=CARTESIAN_POINT ( 'NONE',  ( -102.0695999085541388, -291.3945649229704600, -305.2761892758041427 ) ) ;
#44811=CARTESIAN_POINT ( 'NONE',  ( 35.62967047056401526, -291.7493174923444030, -248.0477402503465498 ) ) ;
#44812=CARTESIAN_POINT ( 'NONE',  ( 36.45533259483765676, -289.1609277709895309, -271.0232163866380120 ) ) ;
#44813=CARTESIAN_POINT ( 'NONE',  ( -92.86785171340416412, -288.0745598828029301, -322.3100952687722156 ) ) ;
#44814=CARTESIAN_POINT ( 'NONE',  ( -39.96089308189817046, -290.5108494771675396, -343.9536993061166186 ) ) ;
#44815=CARTESIAN_POINT ( 'NONE',  ( 34.17068769065854639, -288.5590217795732997, -285.8659523390452364 ) ) ;
#44816=CARTESIAN_POINT ( 'NONE',  ( -25.14856655163930910, -296.8774596948274507, -344.7762146540899266 ) ) ;
#44818=CARTESIAN_POINT ( 'NONE',  ( -37.48536153880243660, -290.2589463793318032, -346.9769168707042013 ) ) ;
#44819=CARTESIAN_POINT ( 'NONE',  ( -81.25936728188860059, -277.4785086805243282, -209.1267704977872484 ) ) ;
#44820=CARTESIAN_POINT ( 'NONE',  ( -112.9762002832144816, -279.0654999807183572, -255.9669613026391914 ) ) ;
#44821=CARTESIAN_POINT ( 'NONE',  ( -42.42441875411951457, -279.6564150252649483, -193.5502446448204239 ) ) ;
#44822=CARTESIAN_POINT ( 'NONE',  ( -110.6135000402559996, -282.7582995383197613, -254.2936281617217844 ) ) ;
#44823=CARTESIAN_POINT ( 'NONE',  ( 128.9467878515196162, -299.5541904835127980, -195.3611179825600175 ) ) ;
#44824=CARTESIAN_POINT ( 'NONE',  ( -13.89668288513848537, -278.4990481378181926, -199.8710056227882319 ) ) ;
#44825=CARTESIAN_POINT ( 'NONE',  ( -109.9454637646575321, -282.3097460895926929, -289.2188602398896933 ) ) ;
#44826=CARTESIAN_POINT ( 'NONE',  ( 121.3887860922853150, -299.5541904835127980, -193.1197964255135844 ) ) ;
#44827=CARTESIAN_POINT ( 'NONE',  ( -109.8844550021252360, -277.3344239351918645, -246.5238099684989095 ) ) ;
#44828=CARTESIAN_POINT ( 'NONE',  ( -109.7125227737370494, -274.1555102275907529, -256.7525563329999159 ) ) ;
#44829=CARTESIAN_POINT ( 'NONE',  ( -85.91723954275585129, -282.6276006684570348, -329.7067958323213475 ) ) ;
#44830=CARTESIAN_POINT ( 'NONE',  ( -87.45133094437605337, -274.1345033083858880, -216.9848356747382070 ) ) ;
#44831=CARTESIAN_POINT ( 'NONE',  ( -67.32131059478003010, -275.0918828034294279, -200.0771991241786054 ) ) ;
#44832=CARTESIAN_POINT ( 'NONE',  ( 32.88152789986077806, -274.9520975295013727, -250.1607706154053119 ) ) ;
#44833=CARTESIAN_POINT ( 'NONE',  ( -64.26376091054356721, -297.4034475821760566, -340.4175866497764105 ) ) ;
#44834=CARTESIAN_POINT ( 'NONE',  ( -1.798836417077152916, -288.7610629285026675, -338.6670829032461825 ) ) ;
#44835=CARTESIAN_POINT ( 'NONE',  ( -31.16659066621182106, -278.2092962448659250, -195.0021606616707288 ) ) ;
#44836=CARTESIAN_POINT ( 'NONE',  ( -114.1126571216632613, -290.3030509816737208, -276.9514797539881670 ) ) ;
#44837=CARTESIAN_POINT ( 'NONE',  ( -110.0244992001172477, -289.4928306369570805, -279.3399356704422303 ) ) ;
#44838=CARTESIAN_POINT ( 'NONE',  ( 36.36459098178308835, -291.3739008404184574, -256.4908871948564411 ) ) ;
#44841=CARTESIAN_POINT ( 'NONE',  ( -108.1665842616880440, -290.2969794809960717, -252.3707939916815519 ) ) ;
#44843=CARTESIAN_POINT ( 'NONE',  ( -23.83911004664717836, -287.1617319711425580, -194.7392162161667954 ) ) ;
#44844=CARTESIAN_POINT ( 'NONE',  ( -102.0172624299486870, -292.6233781216987495, -301.5434626090942061 ) ) ;
#44845=CARTESIAN_POINT ( 'NONE',  ( -70.71644438930614740, -294.5402841608669746, -339.5055105387589833 ) ) ;
#44846=CARTESIAN_POINT ( 'NONE',  ( -13.55923351420843304, -284.0648632846011310, -343.0776398579266697 ) ) ;
#44847=CARTESIAN_POINT ( 'NONE',  ( -102.2374226790117575, -284.8399235084859242, -236.9314126432019521 ) ) ;
#44848=CARTESIAN_POINT ( 'NONE',  ( 36.13560834171039460, -276.8473382598899661, -268.8351374350356764 ) ) ;
#44849=CARTESIAN_POINT ( 'NONE',  ( 24.72254015447936126, -291.0090541605105727, -228.8897196343893370 ) ) ;
#44850=CARTESIAN_POINT ( 'NONE',  ( -6.347422214351442271, -273.2635757185508396, -203.8292816731760979 ) ) ;
#44853=CARTESIAN_POINT ( 'NONE',  ( 21.34877672232704526, -293.8905051744324055, -320.1724843428212353 ) ) ;
#44854=CARTESIAN_POINT ( 'NONE',  ( -71.86739548078840301, -287.5121820922828419, -204.4119666553180821 ) ) ;
#44855=CARTESIAN_POINT ( 'NONE',  ( -114.0013770531242443, -297.6769958988410849, -266.7635474953483481 ) ) ;
#44856=CARTESIAN_POINT ( 'NONE',  ( -30.53003536021292774, -286.7918340046165326, -197.5263639791413368 ) ) ;
#44857=CARTESIAN_POINT ( 'NONE',  ( -112.5654737403736334, -277.4181082703252628, -285.7298566160930591 ) ) ;
#44858=CARTESIAN_POINT ( 'NONE',  ( 13.20522743624334794, -293.3888403381756689, -212.4100964203909427 ) ) ;
#44859=CARTESIAN_POINT ( 'NONE',  ( 37.75417510060062654, -285.5640550156600739, -260.3154719736058382 ) ) ;
#44860=CARTESIAN_POINT ( 'NONE',  ( 37.73973963241286356, -293.6722737940024786, -253.3161059073749186 ) ) ;
#44861=CARTESIAN_POINT ( 'NONE',  ( -33.51157017901221025, -292.4349377721255223, -197.4279968699894141 ) ) ;
#44864=CARTESIAN_POINT ( 'NONE',  ( 161.2402580060632147, 217.6105062135258095, -202.4543169503909610 ) ) ;
#44865=CARTESIAN_POINT ( 'NONE',  ( 25.77291357601318822, -288.5013954184609020, -227.4512683872464152 ) ) ;
#44866=CARTESIAN_POINT ( 'NONE',  ( -19.11405058567864046, -280.3380690714490129, -350.3683826091709648 ) ) ;
#44868=CARTESIAN_POINT ( 'NONE',  ( -95.36951592401595690, -282.8441847773926270, -315.1811527220429525 ) ) ;
#44869=CARTESIAN_POINT ( 'NONE',  ( -113.6955703002261089, -278.3464054398949656, -260.1664551931082769 ) ) ;
#44870=CARTESIAN_POINT ( 'NONE',  ( 35.85318259912133243, -283.3511463421290273, -254.7265447461116139 ) ) ;
#44871=CARTESIAN_POINT ( 'NONE',  ( 7.677621891900887618, -59.82691858394279905, -353.2347412010317385 ) ) ;
#44872=CARTESIAN_POINT ( 'NONE',  ( -102.4257697418197353, -282.5996320843825060, -310.3944812501870274 ) ) ;
#44873=CARTESIAN_POINT ( 'NONE',  ( -27.59742183241397129, -284.1966481620742684, -196.3550652468307192 ) ) ;
#44874=CARTESIAN_POINT ( 'NONE',  ( 13.12379576613483323, -276.6085234987818353, -213.7796218371169630 ) ) ;
#44875=CARTESIAN_POINT ( 'NONE',  ( -49.97071242924983636, -298.3789930052282671, -198.3993469524838531 ) ) ;
#44876=CARTESIAN_POINT ( 'NONE',  ( -4.128678093487827994, -293.2895897531827814, -335.9354004423030347 ) ) ;
#44877=CARTESIAN_POINT ( 'NONE',  ( -98.50033958787030031, -279.8260141020185756, -223.7249293083094983 ) ) ;
#44878=CARTESIAN_POINT ( 'NONE',  ( 11.74770313617410444, -276.3479567014632607, -324.4596143623290914 ) ) ;
#44879=CARTESIAN_POINT ( 'NONE',  ( -113.2404333110514045, -273.7744271896679606, -259.0041579536853078 ) ) ;
#44880=CARTESIAN_POINT ( 'NONE',  ( -25.82999229414716069, -275.8291290068479498, -346.1831008886371706 ) ) ;
#44881=CARTESIAN_POINT ( 'NONE',  ( -95.79658185063551912, -239.9132554249223972, -341.7037225619939136 ) ) ;
#44882=CARTESIAN_POINT ( 'NONE',  ( -18.63779021769444100, -274.8112331595512501, -343.0443770915891264 ) ) ;
#44883=CARTESIAN_POINT ( 'NONE',  ( -76.76256789907030509, -296.9938775006589822, -335.8795331689473187 ) ) ;
#44886=CARTESIAN_POINT ( 'NONE',  ( -67.90074174454966283, -284.5426918370051226, -336.9972271879709638 ) ) ;
#44887=CARTESIAN_POINT ( 'NONE',  ( -83.25287784326982887, -285.4310989093687567, -330.9758397337648717 ) ) ;
#44888=CARTESIAN_POINT ( 'NONE',  ( -74.76517734613999266, -284.8882149780384907, -207.5648121906982908 ) ) ;
#44889=CONICAL_SURFACE ( 'NONE', #4024, 2.241321557046427326, 0.09862129276975473147 ) ;
#44890=CARTESIAN_POINT ( 'NONE',  ( -110.2858528267710625, -276.8057861783671001, -281.5678571466028757 ) ) ;
#44891=CARTESIAN_POINT ( 'NONE',  ( -85.64790207335592243, -285.5894491232702421, -326.7293389164128712 ) ) ;
#44892=CARTESIAN_POINT ( 'NONE',  ( -87.99325395927627369, -277.8083621993210386, -216.7637254420216379 ) ) ;
#44893=CARTESIAN_POINT ( 'NONE',  ( -32.38598643313268610, -278.0680181076066333, -343.5527132183279946 ) ) ;
#44895=CARTESIAN_POINT ( 'NONE',  ( -78.89521878112562092, -273.9677917405644507, -210.2056212678602094 ) ) ;
#44896=CARTESIAN_POINT ( 'NONE',  ( 26.14142257911781186, -281.7817514731621600, -226.9779743120037665 ) ) ;
#44897=CARTESIAN_POINT ( 'NONE',  ( -41.55948849069151407, -283.5961418111362491, -347.2361675200016293 ) ) ;
#44901=CARTESIAN_POINT ( 'NONE',  ( 36.62432930176822765, -289.6219083200477939, -286.8317652917231726 ) ) ;
#44902=CARTESIAN_POINT ( 'NONE',  ( -70.53168554395965373, -296.8000967899567968, -205.1472791797875743 ) ) ;
#44903=CARTESIAN_POINT ( 'NONE',  ( -74.62220758075554272, -290.9180136745612231, -203.1043224092960884 ) ) ;
#44904=CARTESIAN_POINT ( 'NONE',  ( 35.81013993305315068, -286.1485499826483192, -279.2782950993930058 ) ) ;
#44905=CARTESIAN_POINT ( 'NONE',  ( -31.84531552763532858, -287.5563022883413851, -343.7958308776430840 ) ) ;
#44906=CARTESIAN_POINT ( 'NONE',  ( -32.06294684805041584, -290.3594754125659847, -196.5234704348577282 ) ) ;
#44907=CARTESIAN_POINT ( 'NONE',  ( -6.865557171864504760, -287.6663669500873084, -203.5765519488274720 ) ) ;
#44908=CARTESIAN_POINT ( 'NONE',  ( -103.2310110255232303, -276.0760238941593343, -306.1884728315868642 ) ) ;
#44909=CARTESIAN_POINT ( 'NONE',  ( 38.90169518151787287, -285.9671659966109587, -271.5592601806049515 ) ) ;
#44910=CARTESIAN_POINT ( 'NONE',  ( 22.25623811635489346, -288.9287967970451518, -224.8089114094292142 ) ) ;
#44911=CARTESIAN_POINT ( 'NONE',  ( -97.57567154493682438, -287.9389745409797001, -315.3479219858205624 ) ) ;
#44912=CARTESIAN_POINT ( 'NONE',  ( -18.66409561926110072, -283.7470383120365796, -341.2272200174068644 ) ) ;
#44913=CARTESIAN_POINT ( 'NONE',  ( -112.1840283378751195, -292.6485916650241279, -262.8461942793977073 ) ) ;
#44914=CARTESIAN_POINT ( 'NONE',  ( 82.12347693879148380, -301.5478687382300222, -195.3203844934047311 ) ) ;
#44917=CARTESIAN_POINT ( 'NONE',  ( -112.8714614705549621, -298.5173432895429642, -266.8274731023640811 ) ) ;
#44918=CARTESIAN_POINT ( 'NONE',  ( -7.925157689368147906, -279.6448499745104641, -203.3603352654254479 ) ) ;
#44919=CARTESIAN_POINT ( 'NONE',  ( 29.93413013003397793, -279.9906237221798051, -303.6295130106403803 ) ) ;
#44920=CARTESIAN_POINT ( 'NONE',  ( -33.45325553772223515, -294.2015741049136750, -347.1142830203291396 ) ) ;
#44921=CARTESIAN_POINT ( 'NONE',  ( -68.69167761721190857, -271.8742543503462912, -203.3013298842599283 ) ) ;
#44922=CARTESIAN_POINT ( 'NONE',  ( -40.59265452147325703, -275.1731659805272443, -344.7428100305156704 ) ) ;
#44923=CARTESIAN_POINT ( 'NONE',  ( -82.65076559589833494, -297.0010907282301105, -328.2907647318019713 ) ) ;
#44925=CARTESIAN_POINT ( 'NONE',  ( -65.98933895103067471, -272.2593041037410444, -199.5097860267667329 ) ) ;
#44926=CARTESIAN_POINT ( 'NONE',  ( -87.94750118390280136, -293.9878366632519828, -327.1152638649896858 ) ) ;
#44927=CARTESIAN_POINT ( 'NONE',  ( -4.054016701165524594, -296.0295927006360444, -336.0052927053072835 ) ) ;
#44929=CARTESIAN_POINT ( 'NONE',  ( -26.17269284347905867, -295.7091510257329787, -342.6650252273538513 ) ) ;
#44931=CARTESIAN_POINT ( 'NONE',  ( -110.7515609803033811, -282.7896664967382776, -253.3493826984608575 ) ) ;
#44932=CARTESIAN_POINT ( 'NONE',  ( -102.7681588153689631, -296.1118715700067128, -302.8540226837514524 ) ) ;
#44933=CARTESIAN_POINT ( 'NONE',  ( -109.3029549977986647, -284.2036891710071700, -297.9063684378443213 ) ) ;
#44934=CARTESIAN_POINT ( 'NONE',  ( -31.21536424951356281, -282.0489848413953951, -194.9981769272174574 ) ) ;
#44935=CARTESIAN_POINT ( 'NONE',  ( -97.56120596943499379, -284.8610448793852470, -222.4095235575200320 ) ) ;
#44936=CARTESIAN_POINT ( 'NONE',  ( -109.1474470674475157, -288.8244599768494254, -249.2452393417684107 ) ) ;
#44937=CARTESIAN_POINT ( 'NONE',  ( 21.31550574532286291, -272.4094976428775681, -223.6242672951989618 ) ) ;
#44938=CARTESIAN_POINT ( 'NONE',  ( -37.26364556790584004, -284.7379370136624743, -196.8554845851783455 ) ) ;
#44939=CARTESIAN_POINT ( 'NONE',  ( -111.6914943778332230, -289.7093215302534759, -251.5039898923010924 ) ) ;
#44941=CARTESIAN_POINT ( 'NONE',  ( -110.5960206018325920, -298.0300692622855081, -279.7273716327206330 ) ) ;
#44942=CARTESIAN_POINT ( 'NONE',  ( -112.2126018767962989, -279.7842497935694723, -285.6885487601256841 ) ) ;
#44943=CARTESIAN_POINT ( 'NONE',  ( -47.43672265507717611, -293.1999635024898225, -345.0370667288032678 ) ) ;
#44944=CARTESIAN_POINT ( 'NONE',  ( 35.70862955333024757, -281.1954758924251792, -268.5872965196671203 ) ) ;
#44945=CARTESIAN_POINT ( 'NONE',  ( 17.56303478610158564, -294.4606738631777603, -324.4227896493760568 ) ) ;
#44946=CARTESIAN_POINT ( 'NONE',  ( -101.2865750478492970, -283.1691899289404546, -230.1073334596489701 ) ) ;
#44947=CARTESIAN_POINT ( 'NONE',  ( -74.05182509965642623, -281.5645111741306437, -204.9595325700548472 ) ) ;
#44948=CARTESIAN_POINT ( 'NONE',  ( -63.66472440017997769, -294.4625096249060334, -338.7559594641590479 ) ) ;
#44949=CARTESIAN_POINT ( 'NONE',  ( -98.07044248564953648, -271.1552731524466253, -225.9798332660311928 ) ) ;
#44952=CARTESIAN_POINT ( 'NONE',  ( 37.33221743365529477, -283.5082770428304570, -268.5183672133357504 ) ) ;
#44953=CARTESIAN_POINT ( 'NONE',  ( -41.04860782057726709, -294.6076761692886521, -343.3411356771468377 ) ) ;
#44955=CARTESIAN_POINT ( 'NONE',  ( 10.59707575819633618, -273.9094976428776249, -330.5268031993606428 ) ) ;
#44956=CARTESIAN_POINT ( 'NONE',  ( -83.47496131242027673, -272.6351060016030488, -208.8463336005037263 ) ) ;
#44957=CARTESIAN_POINT ( 'NONE',  ( -110.3677456655047138, -290.4105546439384398, -268.4596414602061145 ) ) ;
#44958=CARTESIAN_POINT ( 'NONE',  ( -59.96471228920603380, -281.2738750558607421, -200.1723814198369382 ) ) ;
#44959=CARTESIAN_POINT ( 'NONE',  ( -92.63087372674183939, -274.8430728556506324, -221.4781178799393899 ) ) ;
#44960=CARTESIAN_POINT ( 'NONE',  ( -64.94321019922705318, -285.0068630810242212, -341.4004993741073122 ) ) ;
#44961=CARTESIAN_POINT ( 'NONE',  ( -24.79349950775172928, -279.0107329556851141, -198.0446387747937251 ) ) ;
#44962=CARTESIAN_POINT ( 'NONE',  ( 21.60989744357675946, -278.1890651969129067, -316.7467717988959635 ) ) ;
#44964=CARTESIAN_POINT ( 'NONE',  ( -70.12984044125136052, -273.4653903228503395, -200.6764969470301310 ) ) ;
#44965=CARTESIAN_POINT ( 'NONE',  ( 11.86470794584511168, -294.6617638169417432, -214.4350054671125747 ) ) ;
#44968=CARTESIAN_POINT ( 'NONE',  ( 21.31505990980102538, -292.3461877180073429, -318.3365593364886195 ) ) ;
#44969=CARTESIAN_POINT ( 'NONE',  ( -110.4030052300476115, -272.0958164305236551, -267.6287084019114104 ) ) ;
#44971=CARTESIAN_POINT ( 'NONE',  ( 1.331857138137925389, -294.0786443404025476, -204.5203201921196126 ) ) ;
#44972=CARTESIAN_POINT ( 'NONE',  ( -112.3417001280813849, -275.0519495502701943, -270.3929463913696054 ) ) ;
#44973=CARTESIAN_POINT ( 'NONE',  ( 35.48883471264535672, -289.3302962816950412, -253.1086760576881147 ) ) ;
#44974=CARTESIAN_POINT ( 'NONE',  ( 37.41998447263363659, -273.4966165216893046, -266.0583256298650099 ) ) ;
#44975=CARTESIAN_POINT ( 'NONE',  ( 35.78357977591105765, -277.2921194104836786, -256.4324554781686629 ) ) ;
#44976=CARTESIAN_POINT ( 'NONE',  ( -12.55129066572806806, -292.8072579743591746, -340.6062287963176800 ) ) ;
#44977=CARTESIAN_POINT ( 'NONE',  ( -14.62111816618705795, -282.2038194188187958, -198.0283185196263389 ) ) ;
#44979=CARTESIAN_POINT ( 'NONE',  ( -51.02602017184861438, -282.8984557946668588, -342.1401583220393263 ) ) ;
#44980=CARTESIAN_POINT ( 'NONE',  ( -100.2042186998935165, -279.0487491537156757, -314.2905644712399749 ) ) ;
#44982=CARTESIAN_POINT ( 'NONE',  ( -19.02827411831646032, -281.6165672692053477, -344.7974214811313800 ) ) ;
#44983=CARTESIAN_POINT ( 'NONE',  ( -101.8926164392937892, -278.9455216463430247, -312.0032410400955882 ) ) ;
#44984=CARTESIAN_POINT ( 'NONE',  ( -3.019465798492313002, -278.1271277400308009, -338.5276424403434135 ) ) ;
#44985=CARTESIAN_POINT ( 'NONE',  ( -37.37352853689063181, -282.5519495502701375, -200.3611179825600459 ) ) ;
#44987=CARTESIAN_POINT ( 'NONE',  ( -109.7736464647251182, -298.8030332313194322, -250.8535645650285062 ) ) ;
#44988=CARTESIAN_POINT ( 'NONE',  ( -101.4004482277824195, -292.1184189522355155, -234.6099001427998871 ) ) ;
#44989=CARTESIAN_POINT ( 'NONE',  ( -109.4148316350069052, -276.3213413071885611, -289.7856004683449100 ) ) ;
#44990=CARTESIAN_POINT ( 'NONE',  ( -101.4343284784878847, -291.7689749532872838, -311.2759018222711802 ) ) ;
#44991=CARTESIAN_POINT ( 'NONE',  ( -91.74347583773356973, -290.5987917589371250, -221.5126990191346010 ) ) ;
#44992=CARTESIAN_POINT ( 'NONE',  ( 37.96456850763826196, -286.8617049278752233, -254.5336483576866158 ) ) ;
#44994=CARTESIAN_POINT ( 'NONE',  ( -109.2089677214262764, -282.7324230716570810, -287.1954419439665003 ) ) ;
#44995=CARTESIAN_POINT ( 'NONE',  ( -109.9231648269188497, -292.6146997664095011, -254.7791904466284336 ) ) ;
#44996=CARTESIAN_POINT ( 'NONE',  ( -70.27506980044306317, -284.0899403070055769, -204.4220786081634458 ) ) ;
#44997=CARTESIAN_POINT ( 'NONE',  ( 36.18031487576281080, -282.8436658394828100, -268.5548571121732380 ) ) ;
#44998=CARTESIAN_POINT ( 'NONE',  ( -70.52647021523173976, -290.4201997297916478, -339.5968794339055989 ) ) ;
#44999=CARTESIAN_POINT ( 'NONE',  ( -59.75847031462780024, -280.2462658141396332, -200.7701734572789576 ) ) ;
#45000=CARTESIAN_POINT ( 'NONE',  ( -11.27386834692455686, -291.1792002377596873, -198.2742817387639036 ) ) ;
#45001=CARTESIAN_POINT ( 'NONE',  ( 20.15909876017686742, -287.6623731904183501, -219.3138034766267594 ) ) ;
#45002=CARTESIAN_POINT ( 'NONE',  ( 39.64099133976078804, -288.0593048627596886, -271.5440799452276224 ) ) ;
#45003=CARTESIAN_POINT ( 'NONE',  ( -49.42361886076759703, -286.0606446342503091, -198.3163748136984168 ) ) ;
#45006=CARTESIAN_POINT ( 'NONE',  ( 18.48916599484682521, -294.7043465154985711, -219.1437393988558142 ) ) ;
#45007=CARTESIAN_POINT ( 'NONE',  ( -71.86657925686228054, -294.1837927747952790, -338.6350588064914291 ) ) ;
#45008=CARTESIAN_POINT ( 'NONE',  ( -36.47537942012152001, -276.0998136476359264, -343.6037965660678424 ) ) ;
#45010=CARTESIAN_POINT ( 'NONE',  ( -46.11000515357697083, -297.2922911212299937, -193.9645891778158386 ) ) ;
#45011=CARTESIAN_POINT ( 'NONE',  ( 28.11113576304865447, -291.5758829128906200, -236.4991330379089902 ) ) ;
#45012=CARTESIAN_POINT ( 'NONE',  ( -93.49883555591291895, -295.4691579200028286, -222.1301165406080997 ) ) ;
#45013=CARTESIAN_POINT ( 'NONE',  ( -93.75482582498300133, -292.4199583252784009, -223.3873681428105442 ) ) ;
#45014=CARTESIAN_POINT ( 'NONE',  ( 25.10399850599438665, -294.1035264581045112, -231.8621619403613749 ) ) ;
#45016=CARTESIAN_POINT ( 'NONE',  ( -64.95430543207319829, -293.4118216271949109, -340.2861789718533601 ) ) ;
#45017=CARTESIAN_POINT ( 'NONE',  ( -102.8666662774895428, -298.0654440227073110, -306.9560002683538187 ) ) ;
#45018=CARTESIAN_POINT ( 'NONE',  ( -90.75618442156434185, -290.7740214440402724, -320.5380686947973459 ) ) ;
#45019=CARTESIAN_POINT ( 'NONE',  ( -31.59645874093947171, -295.3110501249717572, -343.2060235448338403 ) ) ;
#45020=CARTESIAN_POINT ( 'NONE',  ( 11.65469459019522702, -278.3558221822689802, -327.6128437602155827 ) ) ;
#45021=CARTESIAN_POINT ( 'NONE',  ( -99.02030575490984177, -277.8423035465062867, -225.0726038609904265 ) ) ;
#45022=CARTESIAN_POINT ( 'NONE',  ( -71.35024695003625084, -272.9634191520783588, -201.3920558591475185 ) ) ;
#45023=CARTESIAN_POINT ( 'NONE',  ( 21.67221892397924066, -279.0056015145915467, -224.9678051746266476 ) ) ;
#45024=CARTESIAN_POINT ( 'NONE',  ( -59.05448767232898888, -278.1756220060979672, -197.3200660267687852 ) ) ;
#45026=CARTESIAN_POINT ( 'NONE',  ( -110.8672608630167673, -295.2586687192013528, -268.7051849345505730 ) ) ;
#45027=CARTESIAN_POINT ( 'NONE',  ( -89.07483363196955395, -275.3254076992274122, -215.9889488845848575 ) ) ;
#45028=CARTESIAN_POINT ( 'NONE',  ( -27.28435202728121212, -274.8346239058199103, -197.9033645069180238 ) ) ;
#45030=CARTESIAN_POINT ( 'NONE',  ( -106.8402410552994297, -288.9508347281673650, -241.2345045657722267 ) ) ;
#45031=CARTESIAN_POINT ( 'NONE',  ( -112.9249582457598393, -290.7368894666012125, -255.5896734205759344 ) ) ;
#45032=CARTESIAN_POINT ( 'NONE',  ( -49.44964024417996740, -275.8984366418305854, -196.1235108769647582 ) ) ;
#45033=CARTESIAN_POINT ( 'NONE',  ( -87.30590175267187192, -295.3534229674876315, -214.6510921349343164 ) ) ;
#45034=CARTESIAN_POINT ( 'NONE',  ( -21.76872404554887552, -282.0545963758418111, -345.6049963776457048 ) ) ;
#45035=CARTESIAN_POINT ( 'NONE',  ( 0.3351527144970434802, -280.5505321844422610, -335.2690112824063249 ) ) ;
#45037=CARTESIAN_POINT ( 'NONE',  ( -37.53567607646679249, -290.8446289544783667, -196.9517884067832085 ) ) ;
#45038=CARTESIAN_POINT ( 'NONE',  ( -110.8317405842020662, -282.8278344389742074, -259.8692433082197226 ) ) ;
#45042=CARTESIAN_POINT ( 'NONE',  ( 36.89081888944549803, -291.4145776736198741, -259.6590728838539235 ) ) ;
#45043=CARTESIAN_POINT ( 'NONE',  ( -40.52004547041168081, -278.6928795587459149, -344.1052492624293677 ) ) ;
#45044=CARTESIAN_POINT ( 'NONE',  ( -95.02556474304107326, -285.0719612038552668, -320.7652892621512706 ) ) ;
#45045=CARTESIAN_POINT ( 'NONE',  ( -92.11121905872373361, -271.3571875064064329, -218.2882905403421319 ) ) ;
#45046=CARTESIAN_POINT ( 'NONE',  ( -12.02198274293792046, -286.3910893566877007, -201.8927901839605852 ) ) ;
#45047=CARTESIAN_POINT ( 'NONE',  ( 34.07667785116749570, -276.7451721625916434, -252.6187899053837214 ) ) ;
#45048=CARTESIAN_POINT ( 'NONE',  ( -72.91158753461822073, -278.3390957636441954, -334.3081891941630488 ) ) ;
#45049=CARTESIAN_POINT ( 'NONE',  ( -86.97831698256817390, -285.7427942221026456, -326.6550523934734542 ) ) ;
#45054=CARTESIAN_POINT ( 'NONE',  ( -65.60547335084395115, -295.2450061577498559, -342.0004692933496244 ) ) ;
#45055=CARTESIAN_POINT ( 'NONE',  ( 23.31371403259033670, -288.9362955945862268, -226.7680637701012643 ) ) ;
#45057=CARTESIAN_POINT ( 'NONE',  ( -55.63300648810263738, -286.7666405000204577, -350.3538533559490702 ) ) ;
#45058=CARTESIAN_POINT ( 'NONE',  ( -77.31959820859130161, -278.4500164629433812, -204.8530250470102203 ) ) ;
#45059=CARTESIAN_POINT ( 'NONE',  ( -102.5208738600124576, -289.4738042523592867, -230.7864546700232893 ) ) ;
#45060=CARTESIAN_POINT ( 'NONE',  ( -86.20016995144860061, -286.8802959206793730, -215.1244492291654922 ) ) ;
#45061=CARTESIAN_POINT ( 'NONE',  ( -105.3823149106760013, -280.6982198208115733, -241.2329743553731873 ) ) ;
#45062=CARTESIAN_POINT ( 'NONE',  ( 34.52453284190504235, -289.3095206890816371, -296.4738004929021145 ) ) ;
#45063=CARTESIAN_POINT ( 'NONE',  ( 35.70260027967242422, -283.3338264577108134, -253.3455124549539619 ) ) ;
#45064=CARTESIAN_POINT ( 'NONE',  ( 36.49406691238041844, -275.9934369045114977, -292.2543696306888705 ) ) ;
#45065=CARTESIAN_POINT ( 'NONE',  ( -82.92914717370662459, -295.4455451274745315, -211.1886760348594407 ) ) ;
#45066=CARTESIAN_POINT ( 'NONE',  ( -103.4105036632464589, -278.9023045922635333, -230.7111070666566661 ) ) ;
#45067=CARTESIAN_POINT ( 'NONE',  ( -97.27393865318751409, -299.0793475167554334, -226.1871146775593786 ) ) ;
#45069=CARTESIAN_POINT ( 'NONE',  ( -110.4683760289727132, -281.2662352645559167, -253.7030783399848985 ) ) ;
#45070=CARTESIAN_POINT ( 'NONE',  ( -16.03966176233213758, -272.5636453452710271, -197.3668200790013429 ) ) ;
#45072=CARTESIAN_POINT ( 'NONE',  ( -39.69694010020822361, -279.5294636104500228, -197.3250209367067498 ) ) ;
#45073=CARTESIAN_POINT ( 'NONE',  ( 24.99480058169025654, -276.1641458837946175, -225.8171231697601797 ) ) ;
#45074=CARTESIAN_POINT ( 'NONE',  ( 32.96227231253141099, -280.2165964070200630, -239.5362632160081944 ) ) ;
#45075=CARTESIAN_POINT ( 'NONE',  ( -29.03747700862987813, -290.7056084709684001, -343.9071164531536624 ) ) ;
#45076=CARTESIAN_POINT ( 'NONE',  ( 7.462758075997037110, -300.1235921870971310, -194.0430978029753817 ) ) ;
#45077=CARTESIAN_POINT ( 'NONE',  ( -78.00474998966045348, -298.7235478835002027, -205.4417441867235823 ) ) ;
#45078=CARTESIAN_POINT ( 'NONE',  ( 30.38723081137278470, -295.1315086119431044, -238.4140699798435321 ) ) ;
#45079=CARTESIAN_POINT ( 'NONE',  ( 13.13500835329171323, -280.3445444974924499, -325.6072067582007321 ) ) ;
#45080=CARTESIAN_POINT ( 'NONE',  ( 37.12735433239998883, -283.4485485312707169, -268.5241133501003219 ) ) ;
#45081=CARTESIAN_POINT ( 'NONE',  ( -102.1332017961093044, -271.0701969018276145, -233.1909701514428264 ) ) ;
#45082=CARTESIAN_POINT ( 'NONE',  ( -66.46442418998211110, -288.3629186996745943, -337.6916125377663889 ) ) ;
#45083=CARTESIAN_POINT ( 'NONE',  ( 195.4004353698729233, 278.2073661579722739, -125.7789885842296229 ) ) ;
#45085=CARTESIAN_POINT ( 'NONE',  ( -34.70546589103574320, -287.5943666202287545, -346.7264017395094697 ) ) ;
#45086=CARTESIAN_POINT ( 'NONE',  ( -56.07510881051521068, -288.9667453944787781, -340.9909315912261150 ) ) ;
#45088=CARTESIAN_POINT ( 'NONE',  ( -114.0317253597367966, -285.6363934468266734, -269.9970591442449290 ) ) ;
#45089=CARTESIAN_POINT ( 'NONE',  ( 13.50833973054514736, -275.1216850459047691, -217.9553842017454031 ) ) ;
#45090=CARTESIAN_POINT ( 'NONE',  ( 35.99542715519331892, -292.1896969670812609, -247.9299282753309512 ) ) ;
#45091=CARTESIAN_POINT ( 'NONE',  ( -18.93474397697080747, -283.4727574689422340, -345.0785568775221464 ) ) ;
#45092=CARTESIAN_POINT ( 'NONE',  ( 38.10619305724723205, -282.9238836683733211, -258.6030662491696717 ) ) ;
#45093=CARTESIAN_POINT ( 'NONE',  ( 15.74202247268584287, -282.6582080530882877, -326.1093259026982309 ) ) ;
#45094=CARTESIAN_POINT ( 'NONE',  ( 0.4072476377180442864, -280.9030664345736454, -207.7957530287029329 ) ) ;
#45095=CARTESIAN_POINT ( 'NONE',  ( -82.13390479932374433, -293.1952119285919025, -326.4764044574609443 ) ) ;
#45096=CARTESIAN_POINT ( 'NONE',  ( 185.9028033071117250, 263.4317942799772254, -153.4147630842123249 ) ) ;
#45098=CARTESIAN_POINT ( 'NONE',  ( 1.852823970357027950, -278.5270857293184008, -334.1700977949444109 ) ) ;
#45099=CARTESIAN_POINT ( 'NONE',  ( -64.53519957046890454, -182.2411953823292095, -361.8101628955362798 ) ) ;
#45100=CARTESIAN_POINT ( 'NONE',  ( -57.92555012658558411, -297.1277065808350244, -200.2169964387891525 ) ) ;
#45101=CARTESIAN_POINT ( 'NONE',  ( 28.00340991085941766, -292.5269609810044358, -229.6458648847749942 ) ) ;
#45102=CARTESIAN_POINT ( 'NONE',  ( -62.10227321110217957, -183.1506894771875977, -358.8537685376919057 ) ) ;
#45103=CARTESIAN_POINT ( 'NONE',  ( -46.04460757818183936, -296.5185567687674961, -194.4475770690140735 ) ) ;
#45104=CARTESIAN_POINT ( 'NONE',  ( -31.83174353413192037, -287.3814744144756901, -344.0063226517897306 ) ) ;
#45105=CARTESIAN_POINT ( 'NONE',  ( -3.757000792347619189, -296.4646659525153609, -336.5790818086119884 ) ) ;
#45106=CARTESIAN_POINT ( 'NONE',  ( -65.29621206716205961, -286.9942735139140950, -202.3379125434092884 ) ) ;
#45108=CARTESIAN_POINT ( 'NONE',  ( 19.36399297508274842, -295.1996923153037073, -322.1810412333751970 ) ) ;
#45109=CARTESIAN_POINT ( 'NONE',  ( -82.82813988057930032, -284.1857026193267188, -327.6009592705700015 ) ) ;
#45110=CARTESIAN_POINT ( 'NONE',  ( -93.36183478589195772, -296.0637447864519913, -218.0367225798047457 ) ) ;
#45111=CARTESIAN_POINT ( 'NONE',  ( -42.05429359205262330, -292.7969977072485790, -193.6672441497979378 ) ) ;
#45112=CARTESIAN_POINT ( 'NONE',  ( 39.65003539072439054, -294.0437803179181060, -270.3037412548086991 ) ) ;
#45113=CARTESIAN_POINT ( 'NONE',  ( -70.22261759564466388, -291.7729128456326180, -205.1856220425692072 ) ) ;
#45116=CARTESIAN_POINT ( 'NONE',  ( -46.01241218824748813, -299.8037154092144760, -195.0940984342157662 ) ) ;
#45117=CARTESIAN_POINT ( 'NONE',  ( -3.985067533389323291, -273.2772448064072819, -201.3876818897225576 ) ) ;
#45120=CARTESIAN_POINT ( 'NONE',  ( 22.58911660123931142, -275.7071640074176457, -318.6294844103896367 ) ) ;
#45122=CARTESIAN_POINT ( 'NONE',  ( -105.1062881034619210, -271.3420952495238794, -241.0015554501175643 ) ) ;
#45123=CARTESIAN_POINT ( 'NONE',  ( -111.5133269532062030, -280.3727286162280734, -273.4328034817352773 ) ) ;
#45124=CARTESIAN_POINT ( 'NONE',  ( -8.276533417617695676, -274.8070813492064985, -338.6836097568491937 ) ) ;
#45125=CARTESIAN_POINT ( 'NONE',  ( -55.40615617779363333, -299.0197282926562252, -199.1691780537907448 ) ) ;
#45126=CARTESIAN_POINT ( 'NONE',  ( -69.60538474506611806, -274.5578717543543803, -204.6156762861326115 ) ) ;
#45127=CARTESIAN_POINT ( 'NONE',  ( 52.39383663106224986, -300.7580296876250827, -194.1371264346019814 ) ) ;
#45128=CARTESIAN_POINT ( 'NONE',  ( -64.28785766289425396, -271.7224101341118967, -199.9745765261779127 ) ) ;
#45129=CARTESIAN_POINT ( 'NONE',  ( -55.82107744325771392, -295.9477058935856917, -341.1412566901580590 ) ) ;
#45130=CARTESIAN_POINT ( 'NONE',  ( -34.81905062895935288, -290.6591863297728082, -196.8151380928799199 ) ) ;
#45131=DIRECTION ( 'NONE',  ( 0.000000000000000000, 0.000000000000000000, -1.000000000000000000 ) ) ;
#45132=CARTESIAN_POINT ( 'NONE',  ( -1.490841160238415286, -277.0820623854073119, -338.4363911341824291 ) ) ;
#45133=CARTESIAN_POINT ( 'NONE',  ( 29.08516528249147726, -275.3092062763931267, -239.9655620876989701 ) ) ;
#45134=CARTESIAN_POINT ( 'NONE',  ( -110.4497822562913569, -283.5240382705361526, -247.6328437178648869 ) ) ;
#45135=CARTESIAN_POINT ( 'NONE',  ( -83.04969576014880772, -297.6758264022215599, -330.0992282372083650 ) ) ;
#45137=CARTESIAN_POINT ( 'NONE',  ( -22.41692696702421728, -285.4451909607376479, -198.6861297509074120 ) ) ;
#45138=CARTESIAN_POINT ( 'NONE',  ( -55.28970393811566453, -281.2823606132413943, -343.3535667886935698 ) ) ;
#45141=CARTESIAN_POINT ( 'NONE',  ( -74.54171139353850606, -275.7942126176051261, -334.3465317551691669 ) ) ;
#45142=CARTESIAN_POINT ( 'NONE',  ( -40.54947208601370789, -275.6679677826193711, -343.8929667267901209 ) ) ;
#45143=CARTESIAN_POINT ( 'NONE',  ( -85.87190686309902787, -281.3805979028120419, -213.1114240415199674 ) ) ;
#45144=CARTESIAN_POINT ( 'NONE',  ( 36.03957926435236914, -276.7372576975240577, -268.8385089166466742 ) ) ;
#45146=CARTESIAN_POINT ( 'NONE',  ( -15.98186973581476522, -272.7236324264439986, -197.1613009186945362 ) ) ;
#45147=CARTESIAN_POINT ( 'NONE',  ( -103.1998488902101485, -281.0330144565799060, -234.1294651699267888 ) ) ;
#45148=DIRECTION ( 'NONE',  ( 0.000000000000000000, 0.000000000000000000, -1.000000000000000000 ) ) ;
#45149=CARTESIAN_POINT ( 'NONE',  ( -32.42500672069236600, -288.0338125280613326, -194.9483283104614770 ) ) ;
#45151=CARTESIAN_POINT ( 'NONE',  ( -112.0305735846379065, -288.6465747594858158, -262.9945332178206741 ) ) ;
#45153=CARTESIAN_POINT ( 'NONE',  ( -104.8259387609394366, -271.6270037598856675, -241.1268748806968176 ) ) ;
#45154=CARTESIAN_POINT ( 'NONE',  ( -70.75583332890995791, -289.7461448569948743, -204.0711399638371404 ) ) ;
#45155=CARTESIAN_POINT ( 'NONE',  ( 197.9738562182569694, 291.4636489450775798, -54.00000000000003553 ) ) ;
#45157=CARTESIAN_POINT ( 'NONE',  ( -2.137956578368298999, -287.0745336519088937, -338.0619613635256542 ) ) ;
#45158=CARTESIAN_POINT ( 'NONE',  ( -108.3639379111494918, -282.4438314177967868, -297.5229566074983723 ) ) ;
#45159=CARTESIAN_POINT ( 'NONE',  ( -98.29953875658031848, -291.1102732204710719, -230.1053603160897296 ) ) ;
#45160=CARTESIAN_POINT ( 'NONE',  ( 11.68498045918677875, -282.1741220505050478, -215.4816181093974592 ) ) ;
#45161=CARTESIAN_POINT ( 'NONE',  ( 34.86457395050867092, -282.5100915984523340, -282.1448232936455156 ) ) ;
#45162=CARTESIAN_POINT ( 'NONE',  ( -102.3660952171709084, -292.0243634817274483, -308.5462183513867558 ) ) ;
#45163=CARTESIAN_POINT ( 'NONE',  ( -113.0482804226602696, -273.0633504042322102, -256.1387965711674610 ) ) ;
#45164=CARTESIAN_POINT ( 'NONE',  ( -34.74133241795624372, -287.0995648637727982, -345.8763633856726756 ) ) ;
#45165=CARTESIAN_POINT ( 'NONE',  ( 39.31730914938719224, -275.4548428485513796, -262.5803437234296211 ) ) ;
#45166=CARTESIAN_POINT ( 'NONE',  ( -78.17554969086438632, -293.4799359874670586, -207.8755714062629352 ) ) ;
#45168=CARTESIAN_POINT ( 'NONE',  ( 21.27581636871892101, -283.4090924074130839, -223.5744983911110353 ) ) ;
#45169=CARTESIAN_POINT ( 'NONE',  ( -102.0410611639040326, -276.0402284917197449, -308.7257748394039254 ) ) ;
#45171=CARTESIAN_POINT ( 'NONE',  ( -54.39609823113228515, -296.2364642377705763, -196.0941137428946206 ) ) ;
#45172=CARTESIAN_POINT ( 'NONE',  ( -2.858256813195671597, -273.8693321143777553, -205.9034977537036752 ) ) ;
#45173=CARTESIAN_POINT ( 'NONE',  ( -103.4590441213144629, -291.6354102548813216, -302.9065412210857176 ) ) ;
#45174=CARTESIAN_POINT ( 'NONE',  ( -14.78528043257007418, -293.2929906924616716, -200.6860408154362005 ) ) ;
#45175=CARTESIAN_POINT ( 'NONE',  ( -79.91016644144995951, -287.2280987407146426, -209.7515123138486217 ) ) ;
#45176=CARTESIAN_POINT ( 'NONE',  ( -4.871144274710508704, -293.8966889868850672, -201.1927054094255425 ) ) ;
#45177=CARTESIAN_POINT ( 'NONE',  ( 8.623319933707730200, -295.7521033646198134, -331.5208694714384023 ) ) ;
#45178=CARTESIAN_POINT ( 'NONE',  ( 34.90804216963066153, -293.2477622781119635, -259.9220211623784849 ) ) ;
#45179=CARTESIAN_POINT ( 'NONE',  ( 34.95045258370333130, -289.2954485910140647, -250.3900061662970984 ) ) ;
#45180=CARTESIAN_POINT ( 'NONE',  ( 38.42595106142651673, -281.8913462562447307, -284.1552629618122410 ) ) ;
#45181=CARTESIAN_POINT ( 'NONE',  ( -77.41760543113989002, -295.5988218694389502, -206.3046115909482694 ) ) ;
#45182=CARTESIAN_POINT ( 'NONE',  ( -104.0393957065789294, -284.8868602709550828, -231.7788981355775491 ) ) ;
#45183=CARTESIAN_POINT ( 'NONE',  ( 25.15719256819412308, -276.9789252480536561, -229.5476984485566732 ) ) ;
#45184=CARTESIAN_POINT ( 'NONE',  ( -52.15415638363281658, -284.6531892598639502, -198.4742510087044707 ) ) ;
#45185=CARTESIAN_POINT ( 'NONE',  ( 37.60438749050560858, -285.6031122645583764, -274.3428293336386332 ) ) ;
#45186=CARTESIAN_POINT ( 'NONE',  ( -112.4887899456751086, -276.8195169561793705, -260.3078896419380044 ) ) ;
#45188=CARTESIAN_POINT ( 'NONE',  ( -96.62108632582739176, -284.6567839485662716, -227.6321340575879901 ) ) ;
#45189=CARTESIAN_POINT ( 'NONE',  ( -2.584091417435443905, -281.7065309206264487, -202.0828801514105066 ) ) ;
#45190=CARTESIAN_POINT ( 'NONE',  ( -78.02191298294135891, -288.6430846323341370, -335.5225966575035272 ) ) ;
#45191=CARTESIAN_POINT ( 'NONE',  ( 2.128938100842102887, -296.2763321718879297, -333.0320720919074802 ) ) ;
#45192=CARTESIAN_POINT ( 'NONE',  ( -28.67161096172971568, -278.5442133670671865, -346.1192893458318736 ) ) ;
#45193=CARTESIAN_POINT ( 'NONE',  ( 18.55442737433081390, -277.5843618685881324, -322.6001953383675414 ) ) ;
#45194=CARTESIAN_POINT ( 'NONE',  ( -109.4923855583653989, -278.2390031494974210, -281.4642074827985994 ) ) ;
#45195=CARTESIAN_POINT ( 'NONE',  ( -89.41943742115684302, -299.3172587378270464, -216.5492110200560489 ) ) ;
#45196=CARTESIAN_POINT ( 'NONE',  ( 26.52840834090303090, -285.0279146709298743, -231.3657635262516123 ) ) ;
#45197=CARTESIAN_POINT ( 'NONE',  ( -103.0976650903270553, -291.6446608309042858, -308.9698980875317034 ) ) ;
#45198=CARTESIAN_POINT ( 'NONE',  ( -12.91816565755876134, -293.6476051672784138, -339.5356289783023271 ) ) ;
#45200=CARTESIAN_POINT ( 'NONE',  ( 33.79505645823167015, -293.4368859832928820, -286.8979776332712390 ) ) ;
#45201=CARTESIAN_POINT ( 'NONE',  ( -68.21698315878484209, -292.7357517187491567, -200.1456008121224386 ) ) ;
#45202=CARTESIAN_POINT ( 'NONE',  ( -110.2693882551973559, -279.1280336688301986, -276.0951271893612784 ) ) ;
#45204=CARTESIAN_POINT ( 'NONE',  ( -104.0191940012461629, -272.1076835389779376, -232.2159098541459343 ) ) ;
#45205=CARTESIAN_POINT ( 'NONE',  ( 24.61621338543899284, -287.5977422319871835, -224.8141121545608883 ) ) ;
#45207=CARTESIAN_POINT ( 'NONE',  ( -51.67720643867760089, -289.5640194169581605, -345.9933700332452418 ) ) ;
#45208=CARTESIAN_POINT ( 'NONE',  ( -79.32490777258617243, -285.8014683859145180, -210.5537660729611105 ) ) ;
#45210=CARTESIAN_POINT ( 'NONE',  ( 192.1024244148038918, 278.6331814114806207, -125.0969603314121201 ) ) ;
#45211=CARTESIAN_POINT ( 'NONE',  ( -98.16163818206972280, -246.2973920797244887, -331.2694274904645795 ) ) ;
#45212=CARTESIAN_POINT ( 'NONE',  ( -29.70671712946214882, -276.1503186283218838, -343.1741368637249820 ) ) ;
#45213=CARTESIAN_POINT ( 'NONE',  ( -74.18045072629446679, -276.4745726304826121, -333.7419709915359931 ) ) ;
#45214=CARTESIAN_POINT ( 'NONE',  ( -67.52344105919280537, -273.3336134654401803, -199.5458173340413737 ) ) ;
#45215=CARTESIAN_POINT ( 'NONE',  ( 86.16957582609755661, 81.18500878458667103, -299.8392340653068118 ) ) ;
#45216=CARTESIAN_POINT ( 'NONE',  ( -100.0708240539403135, -276.6542903988497528, -314.1601509010688460 ) ) ;
#45217=CARTESIAN_POINT ( 'NONE',  ( -65.21070511493633148, -297.1715164502279549, -341.0666820218505109 ) ) ;
#45218=CARTESIAN_POINT ( 'NONE',  ( -75.01671131628461353, -292.0283216296084561, -207.7034720250236433 ) ) ;
#45219=CARTESIAN_POINT ( 'NONE',  ( -80.54270086535738926, -298.2858554099896651, -206.7531993858468695 ) ) ;
#45220=CARTESIAN_POINT ( 'NONE',  ( -37.25995188159799909, -298.5454960940853653, -193.4218861848133599 ) ) ;
#45221=CARTESIAN_POINT ( 'NONE',  ( -107.6022320872742597, -296.4569541852046086, -290.1716619763398057 ) ) ;
#45224=CARTESIAN_POINT ( 'NONE',  ( -110.0481147711410159, -280.2095909619072813, -290.9303053588366765 ) ) ;
#45225=CARTESIAN_POINT ( 'NONE',  ( -34.48753625672294021, -282.5248316686867156, -347.2466215055856651 ) ) ;
#45226=CARTESIAN_POINT ( 'NONE',  ( -108.2751534594444536, -279.8757811649951464, -251.8003907085040112 ) ) ;
#45227=CARTESIAN_POINT ( 'NONE',  ( -113.3644698981806158, -280.3323564312751159, -268.7780245387174318 ) ) ;
#45228=CARTESIAN_POINT ( 'NONE',  ( -89.72150370778508943, -271.7763627424086508, -218.5242206126879694 ) ) ;
#45231=CARTESIAN_POINT ( 'NONE',  ( -41.05330788521634844, -280.1708210584948802, -197.4555353953860788 ) ) ;
#45232=CARTESIAN_POINT ( 'NONE',  ( 38.76283091420440741, -276.2221955361566756, -259.7658749341599105 ) ) ;
#45233=CARTESIAN_POINT ( 'NONE',  ( 32.84101506552177341, -277.2087980024358558, -243.9151894687832680 ) ) ;
#45234=CARTESIAN_POINT ( 'NONE',  ( 37.01424852486154293, -274.3493631398964681, -288.0185317296443372 ) ) ;
#45237=CARTESIAN_POINT ( 'NONE',  ( 37.16449658841762016, -283.3835796849227222, -258.7436466575366580 ) ) ;
#45238=CARTESIAN_POINT ( 'NONE',  ( -91.78650233036469785, -290.4473968438287557, -221.4714791713576858 ) ) ;
#45239=CARTESIAN_POINT ( 'NONE',  ( 34.76153699912342887, -286.5623655861349448, -243.6321826845998828 ) ) ;
#45240=CARTESIAN_POINT ( 'NONE',  ( -96.74831270752116552, -282.1813059380716027, -314.5066545328163556 ) ) ;
#45241=CARTESIAN_POINT ( 'NONE',  ( 12.30091423030655662, -280.9193401043354470, -324.6840942958812093 ) ) ;
#45242=CARTESIAN_POINT ( 'NONE',  ( 33.65420008368713667, -285.3405648149401941, -247.9376844576008523 ) ) ;
#45244=CARTESIAN_POINT ( 'NONE',  ( -30.23915376342894135, -281.3489422889599041, -197.2578755905713592 ) ) ;
#45245=CARTESIAN_POINT ( 'NONE',  ( -105.0270502363382406, -270.9772121191051042, -238.0548643102111726 ) ) ;
#45246=CARTESIAN_POINT ( 'NONE',  ( -52.77570573118055819, -281.6464738944534361, -345.0356331423077449 ) ) ;
#45247=CARTESIAN_POINT ( 'NONE',  ( 35.16963451458115486, -295.7985704197388941, -289.5211545130006243 ) ) ;
#45249=CARTESIAN_POINT ( 'NONE',  ( -82.20262215928330818, -287.4423929164352671, -209.9842883921245971 ) ) ;
#45251=CARTESIAN_POINT ( 'NONE',  ( -25.27593629765922145, -294.1249765053227634, -195.7706927332011446 ) ) ;
#45252=CARTESIAN_POINT ( 'NONE',  ( 35.78947479807442988, -273.3376967054872466, -253.6653443411174180 ) ) ;
#45253=EDGE_CURVE ( 'NONE', #47701, #52349, #43134, .T. ) ;
#45254=CARTESIAN_POINT ( 'NONE',  ( -59.98945543448800777, -288.5355610431782338, -343.7861682017015141 ) ) ;
#45255=CARTESIAN_POINT ( 'NONE',  ( 31.32248278641987937, -292.3114859966649988, -297.5502463081921860 ) ) ;
#45257=CARTESIAN_POINT ( 'NONE',  ( -108.6546515332806422, -277.0034601100138616, -288.1811759551610521 ) ) ;
#45258=CARTESIAN_POINT ( 'NONE',  ( -106.1149816647575079, -294.3235976247425469, -298.3093062014407337 ) ) ;
#45259=CARTESIAN_POINT ( 'NONE',  ( -104.4915344164712536, -291.4664256507214759, -300.3555002621342283 ) ) ;
#45262=CARTESIAN_POINT ( 'NONE',  ( 38.54538599346576433, -292.1390015054272453, -278.8372595960646549 ) ) ;
#45263=CARTESIAN_POINT ( 'NONE',  ( 25.62276755908332859, -288.6276234087768557, -231.8654529919994332 ) ) ;
#45264=CARTESIAN_POINT ( 'NONE',  ( -99.19301482913152768, -289.3844882588369387, -226.2205597104584740 ) ) ;
#45265=CARTESIAN_POINT ( 'NONE',  ( 17.31619302659392901, -288.2773176330660476, -221.0686912890308804 ) ) ;
#45267=DIRECTION ( 'NONE',  ( 0.000000000000000000, 0.000000000000000000, 1.000000000000000000 ) ) ;
#45268=CARTESIAN_POINT ( 'NONE',  ( 10.22799617783092074, -289.1793204394008399, -326.0134130377272186 ) ) ;
#45269=CARTESIAN_POINT ( 'NONE',  ( -33.49307446567431867, -296.9838493624466764, -345.6308163123198938 ) ) ;
#45271=CARTESIAN_POINT ( 'NONE',  ( -31.83989572058621675, -290.1893869203370286, -346.8184997918723980 ) ) ;
#45272=CARTESIAN_POINT ( 'NONE',  ( -9.446048453272680945, -278.4350352833361626, -200.3594078527704028 ) ) ;
#45273=CARTESIAN_POINT ( 'NONE',  ( -51.30461677501067186, -277.5592812958528270, -346.0630416711411499 ) ) ;
#45274=CARTESIAN_POINT ( 'NONE',  ( -6.235019267237946750, -280.1164900257368799, -199.9329394121948837 ) ) ;
#45275=CARTESIAN_POINT ( 'NONE',  ( -99.83819656525525943, -299.0863136954325796, -229.4504473590564828 ) ) ;
#45276=CARTESIAN_POINT ( 'NONE',  ( -72.08263087683934600, -283.5925013757965871, -203.8925661531843900 ) ) ;
#45277=CARTESIAN_POINT ( 'NONE',  ( -110.5272221829468009, -271.6842131151094577, -270.3500670393695486 ) ) ;
#45278=CARTESIAN_POINT ( 'NONE',  ( -21.91497456255137521, -278.3913552543355650, -197.6937699094292782 ) ) ;
#45279=CARTESIAN_POINT ( 'NONE',  ( -91.02056166489622058, -281.8143853665579854, -322.7403168332483574 ) ) ;
#45281=CARTESIAN_POINT ( 'NONE',  ( -20.29995273181706850, -275.3170959679144971, -344.7946832512226933 ) ) ;
#45282=CARTESIAN_POINT ( 'NONE',  ( -90.89792542045735502, -297.3492718299288526, -321.0551192429788898 ) ) ;
#45283=CARTESIAN_POINT ( 'NONE',  ( -65.15296244275525339, -282.3274957100301776, -341.8457227189608716 ) ) ;
#45284=CARTESIAN_POINT ( 'NONE',  ( -106.2043489005842076, -297.1606414831994698, -295.4369382468241838 ) ) ;
#45285=CARTESIAN_POINT ( 'NONE',  ( -15.00614236063741203, -299.6414511227042112, -193.8493901701033337 ) ) ;
#45286=CARTESIAN_POINT ( 'NONE',  ( -62.03285450581438454, -273.3887881194525562, -201.6411472153219222 ) ) ;
#45287=CARTESIAN_POINT ( 'NONE',  ( 33.43570360707399658, -295.8754012357659349, -295.3272527403886443 ) ) ;
#45288=CARTESIAN_POINT ( 'NONE',  ( 20.57430203005223390, -288.4054981593803859, -321.1228455589242685 ) ) ;
#45289=CARTESIAN_POINT ( 'NONE',  ( -42.31047902625270041, -278.0697983300320857, -194.9646629263701527 ) ) ;
#45290=CARTESIAN_POINT ( 'NONE',  ( -109.8662678751797159, -290.0571767206755567, -296.3878539220891639 ) ) ;
#45291=CARTESIAN_POINT ( 'NONE',  ( -90.77260697509257170, -288.8918211602427846, -320.5205821211498005 ) ) ;
#45292=CARTESIAN_POINT ( 'NONE',  ( 32.57754153347347881, -291.9049435989788890, -297.4959718076015633 ) ) ;
#45295=CARTESIAN_POINT ( 'NONE',  ( -108.4117365732641645, -289.8364762266366483, -287.3033244962084041 ) ) ;
#45297=CARTESIAN_POINT ( 'NONE',  ( -30.91553340198313293, -287.0727096231913151, -193.8526052109661748 ) ) ;
#45298=CARTESIAN_POINT ( 'NONE',  ( -102.0455923789670294, -287.4805209788416391, -239.2376011013261916 ) ) ;
#45299=CARTESIAN_POINT ( 'NONE',  ( -65.52829258352753072, -294.4705592145330115, -341.7779320447328928 ) ) ;
#45300=CARTESIAN_POINT ( 'NONE',  ( 0.6381908120249473182, -283.8720357133968264, -336.7903051716934328 ) ) ;
#45301=CARTESIAN_POINT ( 'NONE',  ( -108.7205108743162327, -284.1828665431768286, -285.7196913973003234 ) ) ;
#45302=CARTESIAN_POINT ( 'NONE',  ( 34.37817999008198910, -277.0783432684659715, -286.4652776280779563 ) ) ;
#45303=CARTESIAN_POINT ( 'NONE',  ( 26.26231454023571388, -291.0444558292219881, -231.1940771457058474 ) ) ;
#45304=CARTESIAN_POINT ( 'NONE',  ( 21.81024513933711972, -273.7415758298365631, -226.9079492056313256 ) ) ;
#45307=CARTESIAN_POINT ( 'NONE',  ( 0.8876039443801369000, -288.4861503455589400, -206.4274523369742838 ) ) ;
#45308=CARTESIAN_POINT ( 'NONE',  ( -103.5897455579518009, -298.1377378446680950, -231.6210984090975273 ) ) ;
#45309=CARTESIAN_POINT ( 'NONE',  ( -70.03545256445691791, -286.2611240578390834, -204.9635837788331116 ) ) ;
#45310=CARTESIAN_POINT ( 'NONE',  ( -109.3812106364152044, -277.9488011015175175, -243.6911362088033286 ) ) ;
#45311=CARTESIAN_POINT ( 'NONE',  ( 6.431390130924254045, -293.2813503129785886, -207.1374724414909565 ) ) ;
#45312=CARTESIAN_POINT ( 'NONE',  ( -2.765125299495188038, -284.6438363744840103, -202.9317207452971559 ) ) ;
#45314=CARTESIAN_POINT ( 'NONE',  ( -19.28811968887323047, -295.1594244674266747, -345.2478843144521647 ) ) ;
#45315=CARTESIAN_POINT ( 'NONE',  ( -44.30644667947097304, -292.2950602546472965, -197.6220482425636931 ) ) ;
#45318=CARTESIAN_POINT ( 'NONE',  ( 201.7602898703401593, 289.7935802246203707, -82.39453363547674769 ) ) ;
#45320=CARTESIAN_POINT ( 'NONE',  ( -106.0631733072216889, -286.5016716867549462, -237.1938619162372959 ) ) ;
#45321=CARTESIAN_POINT ( 'NONE',  ( 36.57525178469694538, -279.4809262143061233, -305.9938812882205070 ) ) ;
#45324=CARTESIAN_POINT ( 'NONE',  ( -26.71148304544562180, -281.8342226617896813, -342.9469328395128400 ) ) ;
#45325=CARTESIAN_POINT ( 'NONE',  ( -114.0224314397881642, -278.3108114621884397, -263.0117211945404847 ) ) ;
#45326=CARTESIAN_POINT ( 'NONE',  ( 37.39821335018235260, -283.6004216167411300, -274.0992668617450363 ) ) ;
#45327=CARTESIAN_POINT ( 'NONE',  ( 204.8861976254081014, 293.2992890834860304, -54.00000000000341061 ) ) ;
#45329=CARTESIAN_POINT ( 'NONE',  ( -38.74010266070690278, -281.6441037679083479, -346.7590941683267829 ) ) ;
#45330=CARTESIAN_POINT ( 'NONE',  ( -30.35272573237195814, -284.1609529146971340, -195.9922780480186475 ) ) ;
#45331=CARTESIAN_POINT ( 'NONE',  ( 20.88612265193818018, -276.7498957291303441, -221.8861126911111228 ) ) ;
#45332=CARTESIAN_POINT ( 'NONE',  ( -40.52692408626661802, -298.5034039385015490, -197.3564852134321654 ) ) ;
#45333=CARTESIAN_POINT ( 'NONE',  ( -53.27248478009627775, -293.9454227737210772, -342.1592126568729100 ) ) ;
#45334=CARTESIAN_POINT ( 'NONE',  ( -112.9638711985142265, -279.0279628279747612, -284.3833336986024278 ) ) ;
#45335=CARTESIAN_POINT ( 'NONE',  ( 22.46583636945384654, -276.1369269143394831, -312.3055003260388958 ) ) ;
#45336=CARTESIAN_POINT ( 'NONE',  ( -111.5228456925401588, -273.8787118613371376, -250.6988033055215226 ) ) ;
#45337=CARTESIAN_POINT ( 'NONE',  ( -75.19563939159630195, -276.4647871765138234, -337.0587325738197819 ) ) ;
#45338=CARTESIAN_POINT ( 'NONE',  ( 102.7371733171515018, 116.6117108516616980, -282.8160689237882366 ) ) ;
#45339=CARTESIAN_POINT ( 'NONE',  ( -62.26366848851381519, -275.3759840907413832, -341.1531895201201792 ) ) ;
#45340=CARTESIAN_POINT ( 'NONE',  ( -34.85549540849656580, -296.4467579933129286, -346.7314334226518326 ) ) ;
#45341=CARTESIAN_POINT ( 'NONE',  ( -95.95921662488163406, -280.4090924074130839, -317.1477375740089997 ) ) ;
#45342=CARTESIAN_POINT ( 'NONE',  ( 122.2132510144744231, 146.9671518294229884, -260.0597590233358574 ) ) ;
#45343=CARTESIAN_POINT ( 'NONE',  ( -108.7231442090566560, -285.4117889738186591, -287.1166838504625503 ) ) ;
#45344=CARTESIAN_POINT ( 'NONE',  ( -44.30374784430958357, -284.8990630343463977, -346.0808320929590423 ) ) ;
#45345=CARTESIAN_POINT ( 'NONE',  ( -95.92031844025744647, -276.3273690398260669, -315.2497122343116303 ) ) ;
#45346=CARTESIAN_POINT ( 'NONE',  ( -110.8384229624914070, -286.5480659844130287, -259.9161568516495890 ) ) ;
#45347=CARTESIAN_POINT ( 'NONE',  ( -27.44628998427068112, -278.6598804190817873, -197.2834946226149668 ) ) ;
#45348=CARTESIAN_POINT ( 'NONE',  ( -9.859778334522250276, -277.7642882091117258, -338.3377473352047673 ) ) ;
#45350=CARTESIAN_POINT ( 'NONE',  ( -62.05640394789998737, -274.2142833789010297, -201.6066864400953875 ) ) ;
#45351=CARTESIAN_POINT ( 'NONE',  ( 17.10146738478125172, -281.6070190068512034, -216.0638285496460185 ) ) ;
#45352=CARTESIAN_POINT ( 'NONE',  ( 10.77963033762923928, -281.1892422867358050, -210.2606409147305158 ) ) ;
#45356=CARTESIAN_POINT ( 'NONE',  ( 11.26667213596453010, -288.5773619600907978, -212.1761412293852516 ) ) ;
#45357=CARTESIAN_POINT ( 'NONE',  ( -88.23073484802083044, -296.5147172052627980, -217.7270274236295791 ) ) ;
#45358=CARTESIAN_POINT ( 'NONE',  ( -77.10943649907028430, -290.8828963689570628, -204.4829958289571721 ) ) ;
#45359=CARTESIAN_POINT ( 'NONE',  ( -3.060934746067260015, -287.0708642305584135, -335.6521006424450206 ) ) ;
#45360=CARTESIAN_POINT ( 'NONE',  ( 31.02592621283743313, -286.4898793797690359, -297.7242367025642693 ) ) ;
#45361=CARTESIAN_POINT ( 'NONE',  ( -52.18414238861056731, -287.0629528568209707, -198.4804362149092753 ) ) ;
#45362=CARTESIAN_POINT ( 'NONE',  ( -100.4288371088549496, -276.0045833872349021, -311.0147015159300281 ) ) ;
#45363=CARTESIAN_POINT ( 'NONE',  ( -41.73501447955607802, -287.5064768702104629, -346.4474516866881117 ) ) ;
#45364=CARTESIAN_POINT ( 'NONE',  ( 0.4902437843262560935, -288.5564003803668811, -205.5870525946830014 ) ) ;
#45365=CARTESIAN_POINT ( 'NONE',  ( -86.21227576637539869, -287.7276120389186076, -327.5407576198914512 ) ) ;
#45366=CARTESIAN_POINT ( 'NONE',  ( -1.125255847982187030, -283.5000870675737588, -334.0146929964590186 ) ) ;
#45367=CARTESIAN_POINT ( 'NONE',  ( -72.59692621455712924, -293.5867174684779002, -203.9605973817307358 ) ) ;
#45370=CARTESIAN_POINT ( 'NONE',  ( -109.8269366098551387, -298.1990455389077397, -291.7422298079723078 ) ) ;
#45371=CARTESIAN_POINT ( 'NONE',  ( 7.248817477734777803, -279.8745120617452358, -212.2945343135737915 ) ) ;
#45372=CARTESIAN_POINT ( 'NONE',  ( 8.381231125308847396, -278.6773768312384618, -210.8444522835007717 ) ) ;
#45373=CARTESIAN_POINT ( 'NONE',  ( -24.94396379846014256, -294.0951829077525872, -346.2468234505490727 ) ) ;
#45374=CARTESIAN_POINT ( 'NONE',  ( -67.12369655905537513, -296.0549657981457017, -202.8234196150576452 ) ) ;
#45375=CARTESIAN_POINT ( 'NONE',  ( -18.67908428978831736, -274.8897727197424388, -342.4237363438489297 ) ) ;
#45376=CARTESIAN_POINT ( 'NONE',  ( -6.543092194914787996, -295.9541643134278956, -337.0895918812256582 ) ) ;
#45378=CARTESIAN_POINT ( 'NONE',  ( -37.58583968854548374, -296.5290322190484176, -194.0548393963825049 ) ) ;
#45379=CARTESIAN_POINT ( 'NONE',  ( -108.8890936950013497, -295.1193790189228707, -244.7692347713699519 ) ) ;
#45380=CARTESIAN_POINT ( 'NONE',  ( -7.044103201143063764, -293.8829664374374033, -203.2982330228936974 ) ) ;
#45382=CARTESIAN_POINT ( 'NONE',  ( 23.46979387138168960, -293.7913299739117861, -229.6847867250788227 ) ) ;
#45385=CARTESIAN_POINT ( 'NONE',  ( -88.74541761781200933, -283.3554055588260212, -215.1896759589265571 ) ) ;
#45386=CARTESIAN_POINT ( 'NONE',  ( -9.230880848015225126, -294.6741361445097027, -337.7452057936255869 ) ) ;
#45387=CARTESIAN_POINT ( 'NONE',  ( 37.54836979103883721, -281.7766961099754894, -288.3192426046718424 ) ) ;
#45388=CARTESIAN_POINT ( 'NONE',  ( 19.95782821964991172, -282.7945567765212900, -221.0862162384978546 ) ) ;
#45390=CARTESIAN_POINT ( 'NONE',  ( -37.97801149621697192, -285.7111050242172041, -193.3848917857536378 ) ) ;
#45391=CARTESIAN_POINT ( 'NONE',  ( -110.2068935356522985, -288.7721169223410129, -253.2556226922589246 ) ) ;
#45393=CARTESIAN_POINT ( 'NONE',  ( -35.93159539721197149, -281.5146868155068205, -346.6677561198292778 ) ) ;
#45394=CARTESIAN_POINT ( 'NONE',  ( -38.61677816059080470, -284.7206912621533661, -196.8664610464527414 ) ) ;
#45396=CARTESIAN_POINT ( 'NONE',  ( -93.37638247032192851, -288.7549199201504280, -322.7980247665507818 ) ) ;
#45398=CARTESIAN_POINT ( 'NONE',  ( -61.25331234156099214, -296.9678810366415291, -340.2341483074748112 ) ) ;
#45399=CARTESIAN_POINT ( 'NONE',  ( -108.1038782663013365, -279.6084029904442332, -299.1937459700258728 ) ) ;
#45400=CARTESIAN_POINT ( 'NONE',  ( 20.09720686897920316, -292.2441604142200049, -319.1379441269964445 ) ) ;
#45401=CARTESIAN_POINT ( 'NONE',  ( 34.35581212509651294, -281.0354769907095829, -256.4549142522089937 ) ) ;
#45402=CARTESIAN_POINT ( 'NONE',  ( 8.907849977643639505, -294.6037942475798559, -331.9239242823300629 ) ) ;
#45403=CARTESIAN_POINT ( 'NONE',  ( -72.91307199997635280, -283.6648833478634515, -203.6399051195407424 ) ) ;
#45404=CARTESIAN_POINT ( 'NONE',  ( -31.57787329713963942, -278.9796750358146937, -345.1905724855724884 ) ) ;
#45405=CARTESIAN_POINT ( 'NONE',  ( 14.47431131801815773, -293.3602318227935939, -322.1867267386405729 ) ) ;
#45406=CARTESIAN_POINT ( 'NONE',  ( -45.87632707952064948, -295.9437612409752205, -195.8482949895318654 ) ) ;
#45409=CARTESIAN_POINT ( 'NONE',  ( 18.27179841713029873, -282.8353548065690575, -220.5717056173164963 ) ) ;
#45410=CARTESIAN_POINT ( 'NONE',  ( -108.8380507295385513, -296.2588415518927150, -255.2590379625973469 ) ) ;
#45412=CARTESIAN_POINT ( 'NONE',  ( -106.6662871844225293, -275.6237833571633473, -303.7098442033569086 ) ) ;
#45413=CARTESIAN_POINT ( 'NONE',  ( -92.04691142711175189, -272.4920690627170075, -216.4028129959773139 ) ) ;
#45414=CARTESIAN_POINT ( 'NONE',  ( 38.48426874166048606, -288.7391327601870898, -260.1767811132301631 ) ) ;
#45416=CARTESIAN_POINT ( 'NONE',  ( -110.1228250358153247, -290.3028032226767436, -276.6277950747634122 ) ) ;
#45417=CARTESIAN_POINT ( 'NONE',  ( -7.738527266000467364, -281.9674289834452452, -202.8613197309283578 ) ) ;
#45418=CARTESIAN_POINT ( 'NONE',  ( 9.982640443567225574, -276.3166800180622431, -213.6651805570843692 ) ) ;
#45419=CARTESIAN_POINT ( 'NONE',  ( -77.02369962265692038, -278.3027550229815574, -208.5553415596722573 ) ) ;
#45420=CARTESIAN_POINT ( 'NONE',  ( -43.34239183861888733, -279.1281170144687849, -345.1206815714283493 ) ) ;
#45421=ORIENTED_EDGE ( 'NONE', *, *, #57376, .F. ) ;
#45422=CARTESIAN_POINT ( 'NONE',  ( -97.81174707469406826, -273.0230473028275924, -222.6916998320212144 ) ) ;
#45423=CARTESIAN_POINT ( 'NONE',  ( -33.45727403043565573, -294.0215543308391943, -196.0097927622392149 ) ) ;
#45426=CARTESIAN_POINT ( 'NONE',  ( -7.652043227905751976, -290.5767405007836146, -200.6417173057225227 ) ) ;
#45427=CARTESIAN_POINT ( 'NONE',  ( -35.81076516078687177, -297.7385550635263485, -197.3400633275124108 ) ) ;
#45429=CARTESIAN_POINT ( 'NONE',  ( -110.9689653101546583, -292.3261470910621824, -250.2681969408431257 ) ) ;
#45430=CARTESIAN_POINT ( 'NONE',  ( -72.02372285203398405, -285.9805209788416391, -342.4524372437778652 ) ) ;
#45432=CARTESIAN_POINT ( 'NONE',  ( -5.029538327203971093, -288.4785857742228927, -202.8491923921184252 ) ) ;
#45433=CARTESIAN_POINT ( 'NONE',  ( 29.66092597828588140, -273.9942016153243571, -303.8046688338029639 ) ) ;
#45434=CARTESIAN_POINT ( 'NONE',  ( 23.44281826100330690, -276.8838097012996968, -227.3674839435452952 ) ) ;
#45435=CARTESIAN_POINT ( 'NONE',  ( -86.86923170313787068, -289.4370025524622747, -214.7189427761151137 ) ) ;
#45436=CARTESIAN_POINT ( 'NONE',  ( -99.25353038713504361, -280.9998170667708450, -226.6892648562441082 ) ) ;
#45438=CARTESIAN_POINT ( 'NONE',  ( -7.219043887351488387, -281.9948741418995155, -336.9820435281337723 ) ) ;
#45439=CARTESIAN_POINT ( 'NONE',  ( -105.9054158762234152, -280.0768918527389246, -235.8842601998994724 ) ) ;
#45440=CARTESIAN_POINT ( 'NONE',  ( -65.12256794548457606, -282.2021116134155818, -341.7631486531930136 ) ) ;
#45441=CARTESIAN_POINT ( 'NONE',  ( -98.60836983153294000, -278.8753012676129401, -316.6343406940106320 ) ) ;
#45443=CARTESIAN_POINT ( 'NONE',  ( 38.93726004563531973, -277.0463237552338001, -268.3049113418917955 ) ) ;
#45444=CARTESIAN_POINT ( 'NONE',  ( 34.45848030099739390, -284.0519495502702512, -270.3284710469131937 ) ) ;
#45447=CARTESIAN_POINT ( 'NONE',  ( -109.8981155163390611, -298.3076993857250159, -289.4004353956036084 ) ) ;
#45449=CARTESIAN_POINT ( 'NONE',  ( -103.1167475618589577, -291.1950305726215333, -302.7319259384336760 ) ) ;
#45450=CARTESIAN_POINT ( 'NONE',  ( -3.135702224652512360, -274.6180511108425435, -336.7071541350728694 ) ) ;
#45451=CARTESIAN_POINT ( 'NONE',  ( -75.13990664688658683, -291.3088004263742050, -336.2797769341530625 ) ) ;
#45452=CARTESIAN_POINT ( 'NONE',  ( -7.220676772660138631, -291.8066168539365890, -203.7531858684164945 ) ) ;
#45453=CARTESIAN_POINT ( 'NONE',  ( 30.30559247667618550, -287.5355847231087409, -307.1245452848033892 ) ) ;
#45455=CARTESIAN_POINT ( 'NONE',  ( -107.2840283442263427, -283.2633246017062447, -246.6531743785229480 ) ) ;
#45456=CARTESIAN_POINT ( 'NONE',  ( -59.02771209627567117, -291.1960282464961551, -341.4118680977248914 ) ) ;
#45457=CARTESIAN_POINT ( 'NONE',  ( -104.7552833872145754, -282.6352037471804124, -300.1288277159952145 ) ) ;
#45458=CARTESIAN_POINT ( 'NONE',  ( 36.05928883990203104, -282.9155454294988772, -274.0405602370758515 ) ) ;
#45459=CARTESIAN_POINT ( 'NONE',  ( 32.65525296594349669, -288.8971886022393392, -301.8769357547007530 ) ) ;
#45460=CARTESIAN_POINT ( 'NONE',  ( -109.9644671599078265, -278.9332314735262912, -278.8031483391190477 ) ) ;
#45461=CARTESIAN_POINT ( 'NONE',  ( -70.71080952674611808, -290.4167097496552401, -201.4081538796177711 ) ) ;
#45462=CARTESIAN_POINT ( 'NONE',  ( -21.02823705958982003, -287.0591935928943599, -195.2743032764545319 ) ) ;
#45463=CARTESIAN_POINT ( 'NONE',  ( 27.39641412987663571, -288.5914458608899622, -312.0346382350710996 ) ) ;
#45464=CARTESIAN_POINT ( 'NONE',  ( -53.68760389515414744, -283.4343448557227134, -341.5596103751664145 ) ) ;
#45467=CARTESIAN_POINT ( 'NONE',  ( -37.81153215191077521, -293.9067358323311510, -194.5977710222705355 ) ) ;
#45468=CARTESIAN_POINT ( 'NONE',  ( 32.95677424236795616, -292.6255138529586475, -300.6846207049000554 ) ) ;
#45469=CARTESIAN_POINT ( 'NONE',  ( 9.806408841652247688, -275.4427696346846233, -326.4009633426164214 ) ) ;
#45470=CARTESIAN_POINT ( 'NONE',  ( -93.58252795655131706, -296.6173179792022552, -217.8403250770251418 ) ) ;
#45471=CARTESIAN_POINT ( 'NONE',  ( 36.22816785272396345, -291.9657259607729429, -265.2877138855499197 ) ) ;
#45472=CARTESIAN_POINT ( 'NONE',  ( -60.81634480758365413, -295.9833257022187922, -200.1149254197238747 ) ) ;
#45473=CARTESIAN_POINT ( 'NONE',  ( -95.43804753559827247, -292.3853043251716031, -225.5064089325556722 ) ) ;
#45474=CARTESIAN_POINT ( 'NONE',  ( -0.5911293696887359728, -295.6315310635115452, -333.8510845245479004 ) ) ;
#45476=CARTESIAN_POINT ( 'NONE',  ( -80.83221744197234671, -293.6402437757760708, -331.7321535198165066 ) ) ;
#45477=CARTESIAN_POINT ( 'NONE',  ( -109.3684315644258902, -298.8220211762325107, -249.4074323243745823 ) ) ;
#45478=CARTESIAN_POINT ( 'NONE',  ( 31.19055395851106027, -288.1482299247048218, -244.3967453701713168 ) ) ;
#45479=CARTESIAN_POINT ( 'NONE',  ( -12.38658042349540800, -278.7091946457800304, -341.5189435734233712 ) ) ;
#45480=CARTESIAN_POINT ( 'NONE',  ( -97.62597504121067971, -276.7120119533249181, -317.6243692314821487 ) ) ;
#45481=CARTESIAN_POINT ( 'NONE',  ( -78.77963635257771102, -272.8579550380201226, -205.5829563239488493 ) ) ;
#45482=CARTESIAN_POINT ( 'NONE',  ( 14.91855299223730036, -280.3887284966206721, -323.4448021484951141 ) ) ;
#45483=CARTESIAN_POINT ( 'NONE',  ( -99.01440295012493209, -276.3517975608069719, -315.1372864597314560 ) ) ;
#45484=CARTESIAN_POINT ( 'NONE',  ( -106.2625019978786867, -295.5766965628918683, -244.6964534859231719 ) ) ;
#45486=CARTESIAN_POINT ( 'NONE',  ( -51.58943670903502721, -274.5166287149664299, -198.6092223286751164 ) ) ;
#45488=CARTESIAN_POINT ( 'NONE',  ( -109.9637240354653045, -288.3148092801115467, -290.4720217006682219 ) ) ;
#45489=CARTESIAN_POINT ( 'NONE',  ( -98.15960609521329161, -289.9214753919098939, -317.5859241099873884 ) ) ;
#45490=CARTESIAN_POINT ( 'NONE',  ( -101.1758787357383795, -275.0841720462387912, -230.6720002450604738 ) ) ;
#45491=CARTESIAN_POINT ( 'NONE',  ( -103.0899219365449113, -294.0761666370108287, -306.0990495510316123 ) ) ;
#45492=CARTESIAN_POINT ( 'NONE',  ( 11.38229625971367298, -281.5938503460535003, -329.8448683623522584 ) ) ;
#45494=CARTESIAN_POINT ( 'NONE',  ( 13.69608000795611247, -280.3372934617109422, -325.3870031258165341 ) ) ;
#45496=CARTESIAN_POINT ( 'NONE',  ( -97.07562347925731672, -289.9407734637303520, -227.6255677367136059 ) ) ;
#45497=CARTESIAN_POINT ( 'NONE',  ( -111.3287460388996095, -282.6130557288284422, -276.4259770799287708 ) ) ;
#45499=FACE_OUTER_BOUND ( 'NONE', #44198, .T. ) ;
#45500=CARTESIAN_POINT ( 'NONE',  ( -25.05707924998244351, -290.2085090192244934, -196.3211412705609575 ) ) ;
#45501=CARTESIAN_POINT ( 'NONE',  ( 24.36356781804805038, -276.5192291745055968, -230.0725630325194402 ) ) ;
#45502=CARTESIAN_POINT ( 'NONE',  ( -93.13177514333392537, -285.0368290790923993, -322.8729742429882776 ) ) ;
#45503=CARTESIAN_POINT ( 'NONE',  ( 1.695377242281931540, -272.6497519348476999, -205.6662898434930469 ) ) ;
#45504=CARTESIAN_POINT ( 'NONE',  ( -79.30928351290206990, -285.4682408560149156, -210.5686499560788150 ) ) ;
#45505=CARTESIAN_POINT ( 'NONE',  ( 24.48924943086669970, -277.5265145920085388, -310.3588523930935139 ) ) ;
#45506=CARTESIAN_POINT ( 'NONE',  ( 18.43814199061066361, -277.0266233068542761, -317.7025474139956032 ) ) ;
#45507=CARTESIAN_POINT ( 'NONE',  ( -109.7959477539794619, -286.8036344190833802, -250.7908744896595294 ) ) ;
#45509=CARTESIAN_POINT ( 'NONE',  ( -110.7022369792162806, -271.4005444928837960, -270.3464552583088789 ) ) ;
#45510=CARTESIAN_POINT ( 'NONE',  ( -61.59357835053622665, -295.1919222595469137, -343.4979522127525229 ) ) ;
#45511=TOROIDAL_SURFACE ( 'NONE', #27378, 5.343514653206205445, 0.5000000000000000000 ) ;
#45512=CARTESIAN_POINT ( 'NONE',  ( -52.44584541453723858, -287.8376446061049023, -197.2604230830446852 ) ) ;
#45514=CARTESIAN_POINT ( 'NONE',  ( -55.56934967048407970, -289.3380690714490129, -190.3538533559490702 ) ) ;
#45515=CARTESIAN_POINT ( 'NONE',  ( -67.22926379071574843, -278.5896601590897603, -199.7337433422399613 ) ) ;
#45516=CARTESIAN_POINT ( 'NONE',  ( 3.727702009367767300, -290.9944322968904089, -206.1133273080681363 ) ) ;
#45517=CARTESIAN_POINT ( 'NONE',  ( -109.3939081053258917, -285.8693955373045128, -285.8866541636337502 ) ) ;
#45518=CARTESIAN_POINT ( 'NONE',  ( -88.24358142193966614, -281.0880971204780963, -216.5597149117222102 ) ) ;
#45519=CARTESIAN_POINT ( 'NONE',  ( 11.68550559822367418, -288.1422883373899708, -211.6837322850167880 ) ) ;
#45520=CARTESIAN_POINT ( 'NONE',  ( 35.26596656028086585, -283.7943648840376909, -289.2040261545441808 ) ) ;
#45521=CARTESIAN_POINT ( 'NONE',  ( 21.73199087537919283, -276.3834763413260021, -319.7503783106523088 ) ) ;
#45522=CARTESIAN_POINT ( 'NONE',  ( -94.86531623999313467, -295.2319974161572418, -222.7714986767394691 ) ) ;
#45523=CARTESIAN_POINT ( 'NONE',  ( -110.5490224080664206, -278.6876476061310655, -246.3237672694672824 ) ) ;
#45524=CARTESIAN_POINT ( 'NONE',  ( -91.10244640925002102, -299.2016006828159789, -218.7985242846185940 ) ) ;
#45527=CARTESIAN_POINT ( 'NONE',  ( -114.2704648735229114, -281.0519495502701943, -270.3937649182068981 ) ) ;
#45528=CARTESIAN_POINT ( 'NONE',  ( -77.52692868663658032, -295.6585503666685213, -206.1314294800253606 ) ) ;
#45529=DIRECTION ( 'NONE',  ( 0.000000000000000000, 0.000000000000000000, 1.000000000000000000 ) ) ;
#45530=CARTESIAN_POINT ( 'NONE',  ( -76.39400632000348423, -277.0971558784729609, -332.1693527646413600 ) ) ;
#45531=CARTESIAN_POINT ( 'NONE',  ( -27.06506123191228497, -275.3849648292562051, -194.3974945961427068 ) ) ;
#45532=CARTESIAN_POINT ( 'NONE',  ( 37.63312293349971327, -280.8184052323802007, -286.9019539993181525 ) ) ;
#45533=CARTESIAN_POINT ( 'NONE',  ( -10.33372124884548882, -290.4550891440062514, -339.3257673219179651 ) ) ;
#45534=CARTESIAN_POINT ( 'NONE',  ( -62.63365738748202460, -299.2489763132401777, -198.3678915657765742 ) ) ;
#45535=CARTESIAN_POINT ( 'NONE',  ( -104.2485767827878647, -297.2698683459170752, -307.7720448142459873 ) ) ;
#45536=CARTESIAN_POINT ( 'NONE',  ( -2.812418280082969790, -294.5098884634415981, -203.9701763978480642 ) ) ;
#45537=CARTESIAN_POINT ( 'NONE',  ( 18.96799823851717548, -280.2380545079076910, -319.6485027626505939 ) ) ;
#45538=CARTESIAN_POINT ( 'NONE',  ( 24.87285246547894957, -282.9154631487069196, -229.3944512481102436 ) ) ;
#45539=CARTESIAN_POINT ( 'NONE',  ( 97.70547898648123919, -297.8351309912462739, -195.9657595870598072 ) ) ;
#45540=CARTESIAN_POINT ( 'NONE',  ( -110.1675683560323620, -286.4388702932819228, -247.7594187457609962 ) ) ;
#45541=CARTESIAN_POINT ( 'NONE',  ( -29.15218374684615910, -287.8662535896716577, -343.2113609113800408 ) ) ;
#45542=CARTESIAN_POINT ( 'NONE',  ( -112.2161628243665348, -274.5480466014206513, -270.3865304996752457 ) ) ;
#45544=CARTESIAN_POINT ( 'NONE',  ( -23.43711449686069059, -287.4526104916761255, -345.5498203864059974 ) ) ;
#45545=CARTESIAN_POINT ( 'NONE',  ( -10.73831514386218799, -286.0756019894115525, -202.3450335072697897 ) ) ;
#45547=CARTESIAN_POINT ( 'NONE',  ( -95.09286514771430632, -284.9465771351677859, -320.8219488241056183 ) ) ;
#45548=CARTESIAN_POINT ( 'NONE',  ( 34.64578401469587732, -275.7229976875547663, -258.0439336295440285 ) ) ;
#45550=CARTESIAN_POINT ( 'NONE',  ( -13.94761148858195376, -291.2689298221384320, -197.2696940767142451 ) ) ;
#45551=CARTESIAN_POINT ( 'NONE',  ( 32.30359780815243198, -282.6229670549323032, -303.0879064200020139 ) ) ;
#45552=CARTESIAN_POINT ( 'NONE',  ( 37.98654798598295201, -283.2270188642872881, -282.6232919335828910 ) ) ;
#45553=CARTESIAN_POINT ( 'NONE',  ( -10.70536642750085754, -283.0474915632215129, -342.6413612009325789 ) ) ;
#45554=CARTESIAN_POINT ( 'NONE',  ( -6.769419487506960209, -280.4649844485543326, -204.0576869032705929 ) ) ;
#45555=CARTESIAN_POINT ( 'NONE',  ( -102.0172624299487154, -294.4809262143061801, -239.1787733560258289 ) ) ;
#45556=CARTESIAN_POINT ( 'NONE',  ( -21.71499588232236633, -108.4839169218780910, -362.8552879306906220 ) ) ;
#45558=CARTESIAN_POINT ( 'NONE',  ( 28.38897529805340980, -278.0298666294149257, -306.2397041744081889 ) ) ;
#45559=CARTESIAN_POINT ( 'NONE',  ( -78.66963864116488026, -208.0198793462769515, -356.7005032217571738 ) ) ;
#45560=CARTESIAN_POINT ( 'NONE',  ( -95.36492100020704754, -296.5256593477964202, -225.8750241165226385 ) ) ;
#45561=CARTESIAN_POINT ( 'NONE',  ( 29.42535123994730739, -292.5626858866151565, -232.1290927326580515 ) ) ;
#45562=CARTESIAN_POINT ( 'NONE',  ( 202.9738562182569694, 291.9636489450776367, -53.99999999998589573 ) ) ;
#45563=CARTESIAN_POINT ( 'NONE',  ( -87.06496004988078141, -295.9505321715118953, -212.2723867604173051 ) ) ;
#45564=CARTESIAN_POINT ( 'NONE',  ( -104.7870325975018773, -288.5515923591688647, -300.4468319604254702 ) ) ;
#45565=CARTESIAN_POINT ( 'NONE',  ( -70.25069252932814834, -297.3509958966904492, -336.9033128876343426 ) ) ;
#45566=CARTESIAN_POINT ( 'NONE',  ( 29.24977685218440371, -288.4502730639962351, -239.2674100956153325 ) ) ;
#45568=CARTESIAN_POINT ( 'NONE',  ( -0.9260767199387287540, -293.4648587388385295, -202.7835878029266325 ) ) ;
#45569=CARTESIAN_POINT ( 'NONE',  ( -71.43204248231860731, -284.0076091134063745, -334.9818344748679806 ) ) ;
#45570=CARTESIAN_POINT ( 'NONE',  ( -75.56837538139504318, -296.3492994282260042, -203.9170414095896149 ) ) ;
#45571=CARTESIAN_POINT ( 'NONE',  ( -36.39065828649177803, -292.8666198832204373, -193.5154746173393221 ) ) ;
#45572=CARTESIAN_POINT ( 'NONE',  ( 23.05585864486166869, -293.4062756309799056, -222.6781143594909338 ) ) ;
#45573=CARTESIAN_POINT ( 'NONE',  ( -84.68341567097189682, -289.8923715197121851, -325.9954713532284245 ) ) ;
#45576=CARTESIAN_POINT ( 'NONE',  ( -72.72520418568217337, -299.4494606519844524, -203.3083307234081758 ) ) ;
#45577=CARTESIAN_POINT ( 'NONE',  ( -64.74363624956751551, -272.4971015828929808, -198.8128007990508479 ) ) ;
#45578=CARTESIAN_POINT ( 'NONE',  ( 20.35897310022778228, -281.2445800340760798, -315.4614589779540097 ) ) ;
#45580=CARTESIAN_POINT ( 'NONE',  ( -67.69010906387433124, -276.9475107146832897, -341.0611956234716899 ) ) ;
#45581=CARTESIAN_POINT ( 'NONE',  ( -99.94848574848113287, -271.4855134177338982, -231.2864355309620237 ) ) ;
#45582=CARTESIAN_POINT ( 'NONE',  ( -110.2520349925624146, -280.2305774530794906, -284.3905712111647972 ) ) ;
#45583=CARTESIAN_POINT ( 'NONE',  ( -48.82184626111737202, -275.3393451219001236, -343.7555340053512509 ) ) ;
#45585=CARTESIAN_POINT ( 'NONE',  ( -88.41299835021102638, -298.5223020756208143, -217.5753179060691025 ) ) ;
#45586=CARTESIAN_POINT ( 'NONE',  ( -36.74615914089810786, -275.0010696616401447, -197.1157895607177579 ) ) ;
#45587=CARTESIAN_POINT ( 'NONE',  ( -34.10992547473529868, -299.6920951693327311, -194.1602496597243714 ) ) ;
#45589=CARTESIAN_POINT ( 'NONE',  ( 27.10913097588206355, -273.0503477253616325, -231.2165018471380620 ) ) ;
#45590=CARTESIAN_POINT ( 'NONE',  ( 34.31476452488585238, -294.0130126873669383, -255.8958581531105096 ) ) ;
#45591=CARTESIAN_POINT ( 'NONE',  ( 33.19907940913238775, -291.8496140260870675, -249.2241389348397718 ) ) ;
#45593=ADVANCED_FACE ( 'NONE', ( #80043 ), #75354, .F. ) ;
#45594=CARTESIAN_POINT ( 'NONE',  ( 19.83567369699905569, -276.7440212757485938, -321.8616561260699314 ) ) ;
#45595=CARTESIAN_POINT ( 'NONE',  ( 23.79233879896182202, -275.1660055240000133, -230.4658890827383857 ) ) ;
#45598=CARTESIAN_POINT ( 'NONE',  ( -95.90371218205980597, -282.5696191288851082, -319.6133856714011472 ) ) ;
#45599=CARTESIAN_POINT ( 'NONE',  ( -32.11396708536629774, -296.9865349880702183, -345.3587169459429447 ) ) ;
#45601=CARTESIAN_POINT ( 'NONE',  ( -91.63419927090286876, -284.4508091940504073, -221.2466430781530278 ) ) ;
#45602=CARTESIAN_POINT ( 'NONE',  ( -73.41899128812953279, -281.5290120294010876, -336.3620371340252859 ) ) ;
#45603=CARTESIAN_POINT ( 'NONE',  ( 32.65307508127736469, -274.4258757261377468, -293.0790923753674520 ) ) ;
#45604=CARTESIAN_POINT ( 'NONE',  ( 24.69688571741018634, -282.9815485281977772, -228.1932928273363927 ) ) ;
#45605=CARTESIAN_POINT ( 'NONE',  ( 7.561795982442758302, -275.8857644787175332, -212.3024705588175607 ) ) ;
#45608=CARTESIAN_POINT ( 'NONE',  ( -60.60727323487409279, -272.1552965188378153, -197.7446938302877584 ) ) ;
#45609=CARTESIAN_POINT ( 'NONE',  ( -53.39439349756933950, -281.8470233089592512, -196.8752943729790275 ) ) ;
#45611=CARTESIAN_POINT ( 'NONE',  ( -57.39770104258494854, -287.7155760488382725, -197.4571499221765976 ) ) ;
#45613=CARTESIAN_POINT ( 'NONE',  ( -78.96141488463774749, -289.4913040063623271, -207.9071417150786658 ) ) ;
#45615=CARTESIAN_POINT ( 'NONE',  ( -96.73873518117028425, -294.7466845591411584, -313.5001213031345060 ) ) ;
#45616=CARTESIAN_POINT ( 'NONE',  ( -59.07296906801516201, -287.4757954551026842, -341.3980409767154356 ) ) ;
#45617=CARTESIAN_POINT ( 'NONE',  ( -104.5266604826868644, -260.4492150524036447, -315.3738353148558531 ) ) ;
#45618=CARTESIAN_POINT ( 'NONE',  ( 28.11386210744392855, -285.5147603550024087, -231.0382941334338227 ) ) ;
#45619=CARTESIAN_POINT ( 'NONE',  ( -45.71016593656803195, -284.7599787550973929, -343.7366713543623860 ) ) ;
#45620=CARTESIAN_POINT ( 'NONE',  ( -68.78783806396161538, -281.6997171945549781, -339.5498661768355646 ) ) ;
#45621=CARTESIAN_POINT ( 'NONE',  ( -49.68872445679357241, -291.8904214331853382, -198.3615401739482422 ) ) ;
#45622=CARTESIAN_POINT ( 'NONE',  ( 3.012051695335717039, -282.0305610147144080, -208.7617864277644628 ) ) ;
#45623=CARTESIAN_POINT ( 'NONE',  ( 34.39102420502452162, -282.5452018680484798, -284.8123269644436846 ) ) ;
#45624=CARTESIAN_POINT ( 'NONE',  ( -73.61300428380712901, -291.5108948859240172, -336.4273373719661322 ) ) ;
#45625=CARTESIAN_POINT ( 'NONE',  ( -62.84704857234799391, -297.8957525566902405, -197.7079886264569097 ) ) ;
#45626=CARTESIAN_POINT ( 'NONE',  ( 19.47367773497335008, -286.3190012204545951, -320.1935226074151046 ) ) ;
#45627=CARTESIAN_POINT ( 'NONE',  ( 23.63284201288958641, -274.9243643140495124, -223.3172659238111066 ) ) ;
#45628=CARTESIAN_POINT ( 'NONE',  ( 23.12255955888526771, -294.9329017549430887, -226.5681673112793248 ) ) ;
#45630=CARTESIAN_POINT ( 'NONE',  ( 10.59707575819634329, -289.1948066931273615, -210.1954327657594490 ) ) ;
#45631=CARTESIAN_POINT ( 'NONE',  ( -87.99589381103636754, -275.7586119622723686, -325.8965218836639792 ) ) ;
#45633=CARTESIAN_POINT ( 'NONE',  ( -34.77229958908775131, -296.4836907700839106, -194.1617984748187951 ) ) ;
#45634=CARTESIAN_POINT ( 'NONE',  ( -108.1687548953238718, -292.4241675039580173, -249.5805152551563424 ) ) ;
#45635=CARTESIAN_POINT ( 'NONE',  ( -92.98598755200396226, -272.5743308168722479, -222.9328754195846045 ) ) ;
#45636=CARTESIAN_POINT ( 'NONE',  ( -98.88916998517707668, -292.6301500274031469, -229.7391823582665609 ) ) ;
#45637=CARTESIAN_POINT ( 'NONE',  ( -79.67645885818227214, -292.4057722322374957, -210.5396295467203629 ) ) ;
#45638=CARTESIAN_POINT ( 'NONE',  ( -101.2652043455636317, -285.8072700437970184, -307.6674126302619925 ) ) ;
#45639=CARTESIAN_POINT ( 'NONE',  ( -14.06336502786892417, -293.7734700788188320, -197.5269704734126890 ) ) ;
#45640=CARTESIAN_POINT ( 'NONE',  ( -66.84087041418604258, -292.9887558954102929, -199.7700617090935111 ) ) ;
#45641=CARTESIAN_POINT ( 'NONE',  ( -9.232842586139812013, -294.5074830280550486, -337.7460241464402202 ) ) ;
#45642=CARTESIAN_POINT ( 'NONE',  ( 32.35290214813241505, -289.9147606742875496, -298.2080427116193277 ) ) ;
#45643=CARTESIAN_POINT ( 'NONE',  ( 39.64055341967383583, -281.6774875402339831, -267.0552597894484279 ) ) ;
#45644=CARTESIAN_POINT ( 'NONE',  ( -23.66001027692723113, -296.3020032288601442, -194.8055446936759267 ) ) ;
#45645=CARTESIAN_POINT ( 'NONE',  ( -109.0277035254822096, -284.7434153487417348, -242.1071058771530033 ) ) ;
#45646=CARTESIAN_POINT ( 'NONE',  ( 32.65208208140603574, -277.1937960940956032, -244.4243245598644023 ) ) ;
#45648=CARTESIAN_POINT ( 'NONE',  ( -106.9037408604303749, -283.6583135665346731, -246.7872725094422890 ) ) ;
#45649=CARTESIAN_POINT ( 'NONE',  ( 21.44067657335259369, -284.9118906800316608, -223.7613209704549035 ) ) ;
#45650=CARTESIAN_POINT ( 'NONE',  ( -31.15067829409903410, -278.2690247337371261, -194.7978381986755210 ) ) ;
#45653=CARTESIAN_POINT ( 'NONE',  ( -53.70954836035492974, -282.7754236523094846, -341.6177555141230187 ) ) ;
#45654=AXIS2_PLACEMENT_3D ( 'NONE', #31327, #65476, #59758 ) ;
#45655=CARTESIAN_POINT ( 'NONE',  ( -31.12138616649496825, -281.3340218728075683, -193.9587387820884032 ) ) ;
#45656=CARTESIAN_POINT ( 'NONE',  ( 31.47116832282170051, -287.0508315903869061, -304.5046216165504802 ) ) ;
#45657=CARTESIAN_POINT ( 'NONE',  ( -26.03073724693619440, -296.6663055088438341, -343.5050591555380493 ) ) ;
#45658=CARTESIAN_POINT ( 'NONE',  ( -6.875639856457484100, -278.2590755929206239, -340.2197667536778454 ) ) ;
#45659=CARTESIAN_POINT ( 'NONE',  ( 22.26738191377638287, -277.5143925991428091, -318.3407413579136573 ) ) ;
#45660=CARTESIAN_POINT ( 'NONE',  ( -104.2722381377984249, -277.9921105565053381, -299.6305959823988587 ) ) ;
#45661=CARTESIAN_POINT ( 'NONE',  ( -73.76084226763950369, -299.5675580647859988, -204.9877708626372907 ) ) ;
#45662=CARTESIAN_POINT ( 'NONE',  ( 29.30215902541796424, -285.0995438386668184, -236.2082168952213692 ) ) ;
#45664=CARTESIAN_POINT ( 'NONE',  ( -112.0793132728468180, -291.9636826002020484, -285.2841397491514499 ) ) ;
#45665=CARTESIAN_POINT ( 'NONE',  ( -63.69289178503709081, -294.3241125446313617, -338.8242694400125856 ) ) ;
#45667=CARTESIAN_POINT ( 'NONE',  ( 12.36616173313047362, -294.0038836915295519, -323.9207518809613475 ) ) ;
#45668=EDGE_LOOP ( 'NONE', ( #27629, #9379, #623, #71071, #79018 ) ) ;
#45669=CARTESIAN_POINT ( 'NONE',  ( -48.80914246965920000, -290.2744646820648313, -346.2435348289337185 ) ) ;
#45670=CARTESIAN_POINT ( 'NONE',  ( -87.60672713312604287, -279.9795476664357352, -217.2127247687157876 ) ) ;
#45673=CARTESIAN_POINT ( 'NONE',  ( -109.5551561951845798, -295.7997391763244082, -244.5404039696304892 ) ) ;
#45674=CARTESIAN_POINT ( 'NONE',  ( 27.04786786660995901, -287.6505331443672162, -228.3218943935549134 ) ) ;
#45675=CARTESIAN_POINT ( 'NONE',  ( 7.925507525896447802, -288.7859810419243445, -332.6893961040652243 ) ) ;
#45676=CARTESIAN_POINT ( 'NONE',  ( -69.01449666444777620, -283.8138239349079868, -336.1694640855753278 ) ) ;
#45677=CARTESIAN_POINT ( 'NONE',  ( 44.71985729441861679, 12.68782823283341976, -331.8881429784326542 ) ) ;
#45678=CARTESIAN_POINT ( 'NONE',  ( -57.44685790939539061, -168.5996598868645151, -362.8288648292558491 ) ) ;
#45679=CARTESIAN_POINT ( 'NONE',  ( 5.477995611911152807, -59.15194608217792194, -350.9341101783960539 ) ) ;
#45680=CARTESIAN_POINT ( 'NONE',  ( 5.483046864865452008, -275.6530729825468597, -329.7418210916221710 ) ) ;
#45681=CARTESIAN_POINT ( 'NONE',  ( -48.66911171699923244, -276.1199639527063709, -342.8414206653997098 ) ) ;
#45682=CARTESIAN_POINT ( 'NONE',  ( -3.437894570502412428, -297.9736291090912914, -193.4253938243076902 ) ) ;
#45683=CARTESIAN_POINT ( 'NONE',  ( -110.3499271114021809, -272.7333562712346406, -270.3634251448670511 ) ) ;
#45684=CARTESIAN_POINT ( 'NONE',  ( -108.2059980171341493, -276.8683979385705243, -299.1977189667084644 ) ) ;
#45685=CARTESIAN_POINT ( 'NONE',  ( -92.45401980446736445, -290.3604962665202152, -318.4014999859691102 ) ) ;
#45686=CARTESIAN_POINT ( 'NONE',  ( -34.06580258553204743, -298.8950159181937920, -193.5221595209639531 ) ) ;
#45687=CARTESIAN_POINT ( 'NONE',  ( 34.76476796316281082, -286.4240113453520280, -284.6352770580871265 ) ) ;
#45688=CARTESIAN_POINT ( 'NONE',  ( -99.48958076887087998, -273.8064184119138531, -224.9853538378266649 ) ) ;
#45689=CARTESIAN_POINT ( 'NONE',  ( -107.4599590130346627, -296.9874427276698157, -250.0527508532690604 ) ) ;
#45692=CARTESIAN_POINT ( 'NONE',  ( -23.18427210332027499, -278.7927552466910583, -344.6361315474793514 ) ) ;
#45693=CARTESIAN_POINT ( 'NONE',  ( 6.884506129449763812, -281.9759780573676835, -333.3831494306261902 ) ) ;
#45694=CARTESIAN_POINT ( 'NONE',  ( -108.5933385423970918, -279.8584088728788402, -253.1149561518478208 ) ) ;
#45695=CARTESIAN_POINT ( 'NONE',  ( -69.84692176516939810, -279.2343948595678853, -339.0585829547333674 ) ) ;
#45696=CARTESIAN_POINT ( 'NONE',  ( -98.93084734932266144, -295.6816983144295818, -229.9929908724099050 ) ) ;
#45698=CARTESIAN_POINT ( 'NONE',  ( -72.13157725982077295, -279.7450106879030045, -206.1842962033713889 ) ) ;
#45699=CARTESIAN_POINT ( 'NONE',  ( 2.325868589020117394, -275.3722994125948276, -204.5534982684129659 ) ) ;
#45700=CARTESIAN_POINT ( 'NONE',  ( 6.056408941011271807, -276.6406331761798469, -209.1287396833405126 ) ) ;
#45701=CARTESIAN_POINT ( 'NONE',  ( 38.55013076045835874, -274.2445042629233285, -279.6940805236175152 ) ) ;
#45704=CARTESIAN_POINT ( 'NONE',  ( -22.69833766112011730, -291.4415620824499342, -198.6800628696826436 ) ) ;
#45705=CARTESIAN_POINT ( 'NONE',  ( -114.2532078311111121, -283.8697264757878429, -272.8376627250395927 ) ) ;
#45706=CARTESIAN_POINT ( 'NONE',  ( 36.04048113988255864, -279.6615427907082108, -260.3340283629655687 ) ) ;
#45707=CARTESIAN_POINT ( 'NONE',  ( 35.94089608900212340, -280.0320006008110454, -263.1111990805325149 ) ) ;
#45708=CARTESIAN_POINT ( 'NONE',  ( -73.04357601725816096, -283.6550168022467346, -205.0267161194683752 ) ) ;
#45709=CARTESIAN_POINT ( 'NONE',  ( -5.853555897882434245, -290.6383817648881518, -338.4448159084312806 ) ) ;
#45710=CARTESIAN_POINT ( 'NONE',  ( -39.72944173616106411, -281.2266120858207614, -196.9903051133822771 ) ) ;
#45713=CARTESIAN_POINT ( 'NONE',  ( -41.54559616467430061, -281.5040041371852340, -346.4968517232152294 ) ) ;
#45714=CARTESIAN_POINT ( 'NONE',  ( 35.52318391697206579, -295.7811210881617967, -288.1831435745842782 ) ) ;
#45715=CARTESIAN_POINT ( 'NONE',  ( -39.53524766614383879, -278.2648610296914740, -194.3932365179788064 ) ) ;
#45717=CARTESIAN_POINT ( 'NONE',  ( -108.2689656642828879, -278.9697291758607207, -288.1105972686424366 ) ) ;
#45718=CARTESIAN_POINT ( 'NONE',  ( -108.2562835291710712, -286.8743724088337217, -245.4382311826703926 ) ) ;
#45721=CARTESIAN_POINT ( 'NONE',  ( -108.1334674485389229, -292.8144647908335969, -243.7952220366863685 ) ) ;
#45723=CARTESIAN_POINT ( 'NONE',  ( 37.59901702092596310, -273.6044406513971126, -274.4462853850380384 ) ) ;
#45724=CARTESIAN_POINT ( 'NONE',  ( -26.17813813494850805, -288.1106463963140527, -346.3843624788316902 ) ) ;
#45725=CARTESIAN_POINT ( 'NONE',  ( -22.56069930672988377, -290.6443945941650782, -198.0564678708298914 ) ) ;
#45727=CARTESIAN_POINT ( 'NONE',  ( -109.9820225922646699, -277.0906945545703479, -281.5247657138087902 ) ) ;
#45728=CARTESIAN_POINT ( 'NONE',  ( -93.66638592701164612, -295.3688994145142601, -221.9846166831470100 ) ) ;
#45729=CARTESIAN_POINT ( 'NONE',  ( -82.83852812958338063, -291.0047492365516177, -328.0783781251117261 ) ) ;
#45731=CARTESIAN_POINT ( 'NONE',  ( 38.12793609700450759, -292.1742775381973161, -281.6323983360254033 ) ) ;
#45732=CARTESIAN_POINT ( 'NONE',  ( -9.207062669472854566, -288.0263425686655410, -202.1207639795974842 ) ) ;
#45733=CARTESIAN_POINT ( 'NONE',  ( 26.58006272377040347, -286.3393205788928526, -311.5431540319728470 ) ) ;
#45735=CARTESIAN_POINT ( 'NONE',  ( 24.01539413042885585, -288.4171301277321504, -229.6403089738427070 ) ) ;
#45737=CARTESIAN_POINT ( 'NONE',  ( 23.64975031538770978, -288.9146848615072258, -310.7900036098784540 ) ) ;
#45738=CARTESIAN_POINT ( 'NONE',  ( -19.64847687873387017, -296.8057705281709673, -343.6634301530109497 ) ) ;
#45740=CARTESIAN_POINT ( 'NONE',  ( 26.79686661275973236, -288.2041063739244464, -228.4773147319844497 ) ) ;
#45741=CARTESIAN_POINT ( 'NONE',  ( -105.0657823815663789, -276.1918128503554044, -303.9865664869094530 ) ) ;
#45742=CARTESIAN_POINT ( 'NONE',  ( -114.3636775844629909, -278.8697807752670315, -271.6122899129514394 ) ) ;
#45743=CARTESIAN_POINT ( 'NONE',  ( 23.73312251748550494, -280.5934339566821905, -223.4822426775248516 ) ) ;
#45744=CARTESIAN_POINT ( 'NONE',  ( -102.6658987951841624, -299.0147943810757170, -234.2419282270451788 ) ) ;
#45745=CARTESIAN_POINT ( 'NONE',  ( -89.05561611617861217, -283.3248562402314974, -216.0410338509788630 ) ) ;
#45747=CARTESIAN_POINT ( 'NONE',  ( -88.36265214200426499, -277.4681230353219803, -216.3667475058300340 ) ) ;
#45748=CARTESIAN_POINT ( 'NONE',  ( -55.24996249445619867, -281.2823606113562391, -343.1917076044891246 ) ) ;
#45750=CARTESIAN_POINT ( 'NONE',  ( 35.82311797338002179, -274.3069072277313580, -292.0778300268077032 ) ) ;
#45752=CARTESIAN_POINT ( 'NONE',  ( -109.2643544692940054, -297.8624451583949053, -286.4185009329046352 ) ) ;
#45754=CARTESIAN_POINT ( 'NONE',  ( 13.46567483052855785, -281.2811382490925212, -327.8783178160979901 ) ) ;
#45755=CARTESIAN_POINT ( 'NONE',  ( -107.0896943760818800, -297.1962788232704042, -292.8551309309443127 ) ) ;
#45756=CARTESIAN_POINT ( 'NONE',  ( -49.64241171197495817, -275.3236409969477450, -194.8935412771584481 ) ) ;
#45757=CARTESIAN_POINT ( 'NONE',  ( -54.21230415684278370, -273.4961626341039391, -199.3155677603087952 ) ) ;
#45758=CARTESIAN_POINT ( 'NONE',  ( 36.68395610587595712, -295.3965629750618973, -258.2309605837090771 ) ) ;
#45759=CARTESIAN_POINT ( 'NONE',  ( 22.08882082376648626, -287.0610279596776309, -221.4018166811355854 ) ) ;
#45761=CARTESIAN_POINT ( 'NONE',  ( -94.79466800568168594, -277.3067975407060999, -221.2650810117346794 ) ) ;
#45762=CARTESIAN_POINT ( 'NONE',  ( -107.2595396599919439, -290.7995431253098104, -237.9773744700004272 ) ) ;
#45763=CARTESIAN_POINT ( 'NONE',  ( -109.6533385077990346, -289.4573971865952444, -282.0347029890415911 ) ) ;
#45764=CARTESIAN_POINT ( 'NONE',  ( 36.38635201542622610, -291.7294831584885628, -284.1844761798510604 ) ) ;
#45766=CARTESIAN_POINT ( 'NONE',  ( 5.045406874201050940, -57.93311274753654061, -355.0152878038887820 ) ) ;
#45767=CARTESIAN_POINT ( 'NONE',  ( -31.87300104025324288, -288.4890768506405720, -343.2683674209994820 ) ) ;
#45769=CARTESIAN_POINT ( 'NONE',  ( -92.25701923106899471, -284.7553235442392179, -323.9999839339699292 ) ) ;
#45770=CARTESIAN_POINT ( 'NONE',  ( -3.414509733504233591, -291.5478656417370189, -201.4861414817669072 ) ) ;
#45771=CARTESIAN_POINT ( 'NONE',  ( -19.02015581277936818, -284.1364114620302530, -344.6964056223281432 ) ) ;
#45772=CARTESIAN_POINT ( 'NONE',  ( 7.792294985536637242, -282.2495523118050755, -327.8009524001496402 ) ) ;
#45773=CARTESIAN_POINT ( 'NONE',  ( -108.8885982330457693, -296.9147991848542461, -241.7566077735413046 ) ) ;
#45774=CARTESIAN_POINT ( 'NONE',  ( 16.90640573333437757, -277.5739549105646233, -319.9620116658109623 ) ) ;
#45775=CARTESIAN_POINT ( 'NONE',  ( 16.06967236478934780, -290.8338130546777052, -218.1423366041460383 ) ) ;
#45776=CARTESIAN_POINT ( 'NONE',  ( 26.99192173424906116, -273.8658235307314044, -234.9236410926782241 ) ) ;
#45779=CARTESIAN_POINT ( 'NONE',  ( -46.93419291606023336, -287.8496922318884117, -196.4899774052231294 ) ) ;
#45781=CARTESIAN_POINT ( 'NONE',  ( -112.0016977470587562, -297.4109568845370859, -287.9500546963178067 ) ) ;
#45782=CARTESIAN_POINT ( 'NONE',  ( -106.6315861683758754, -285.5145032322628822, -246.9043986513040920 ) ) ;
#45783=CARTESIAN_POINT ( 'NONE',  ( -62.34072999955220240, -276.4281698334281714, -342.9973423688041976 ) ) ;
#45784=CARTESIAN_POINT ( 'NONE',  ( 39.12383935974016680, -294.0954653115360315, -261.7291093873472505 ) ) ;
#45785=CARTESIAN_POINT ( 'NONE',  ( 34.68234878705622748, -285.3891839350876580, -246.6805822762495097 ) ) ;
#45786=CARTESIAN_POINT ( 'NONE',  ( 39.63469959446032931, -293.8488046098257200, -267.4331719496009896 ) ) ;
#45788=CARTESIAN_POINT ( 'NONE',  ( -110.3890624587668583, -290.9104354157870489, -268.4654437844370136 ) ) ;
#45792=CARTESIAN_POINT ( 'NONE',  ( 103.3612552652909073, 114.3676014650440607, -279.5696956816383931 ) ) ;
#45793=CARTESIAN_POINT ( 'NONE',  ( -54.82472594265806265, -287.3514688123764813, -196.0842604881143529 ) ) ;
#45794=CARTESIAN_POINT ( 'NONE',  ( -111.2586520408596868, -270.4809262143062369, -234.7283546768995564 ) ) ;
#45797=CARTESIAN_POINT ( 'NONE',  ( -87.14889238244082037, -282.6857330485477746, -324.2215609949718669 ) ) ;
#45798=CARTESIAN_POINT ( 'NONE',  ( -96.13578908915418708, -277.5490490629295550, -320.0704915305914824 ) ) ;
#45799=CARTESIAN_POINT ( 'NONE',  ( 12.50860946794144901, -282.7489176731266980, -214.5491563876983321 ) ) ;
#45800=CARTESIAN_POINT ( 'NONE',  ( -87.72729469658391110, -231.2803686896094746, -346.7935326881681135 ) ) ;
#45801=CARTESIAN_POINT ( 'NONE',  ( -1.923499357700632295, -281.1670612415235837, -338.0675235028114685 ) ) ;
#45802=CARTESIAN_POINT ( 'NONE',  ( 19.03463836886439964, -284.8902242445822139, -221.4371436695146826 ) ) ;
#45804=CARTESIAN_POINT ( 'NONE',  ( -64.48012981312817260, -275.5620986860499784, -199.6095362881306130 ) ) ;
#45805=CARTESIAN_POINT ( 'NONE',  ( -38.33684707318784746, -295.5573083508033960, -343.4158791170682434 ) ) ;
#45807=CARTESIAN_POINT ( 'NONE',  ( 25.27677249996951758, -291.7090668972056164, -231.7914899641262991 ) ) ;
#45808=CARTESIAN_POINT ( 'NONE',  ( -108.5589040043047362, -278.8346685094983286, -299.3684042804711680 ) ) ;
#45809=CARTESIAN_POINT ( 'NONE',  ( 7.580393323300029351, -276.4197835862396460, -327.9668672037786905 ) ) ;
#45810=CARTESIAN_POINT ( 'NONE',  ( 23.26527609928194096, -275.1027384632600956, -317.3748252414483204 ) ) ;
#45812=CARTESIAN_POINT ( 'NONE',  ( 14.80310999835316466, -274.3177913255401563, -324.3390232105376754 ) ) ;
#45815=CARTESIAN_POINT ( 'NONE',  ( 22.71987118897137492, -295.6141513449050535, -317.6178438562093902 ) ) ;
#45817=CARTESIAN_POINT ( 'NONE',  ( 193.8665746513534316, 275.1768195097669150, -123.9090917457166938 ) ) ;
#45819=CARTESIAN_POINT ( 'NONE',  ( -102.0375808334600833, -285.1626734958675229, -304.9462029551175988 ) ) ;
#45820=CARTESIAN_POINT ( 'NONE',  ( -78.59059452445588079, -285.3596057438592766, -334.1772814792511781 ) ) ;
#45821=CARTESIAN_POINT ( 'NONE',  ( -8.206709036857517958, -285.7926714755894295, -203.3160214985641687 ) ) ;
#45822=CARTESIAN_POINT ( 'NONE',  ( -62.07694774708168239, -275.7789239439487687, -339.9467985368535778 ) ) ;
#45823=CARTESIAN_POINT ( 'NONE',  ( 34.85693152696198638, -283.6372873841950195, -287.6844053778939951 ) ) ;
#45824=CARTESIAN_POINT ( 'NONE',  ( -59.42099449088976826, -275.8231556305547088, -340.6691012535990239 ) ) ;
#45825=CARTESIAN_POINT ( 'NONE',  ( -4.917039185721430172, -277.6945688171628603, -336.1235848688297665 ) ) ;
#45827=CARTESIAN_POINT ( 'NONE',  ( -6.304983870383714439, -281.2524201205200143, -200.0554756385484154 ) ) ;
#45830=CARTESIAN_POINT ( 'NONE',  ( 38.19307660566169460, -281.8613876325513274, -255.7315449472019679 ) ) ;
#45834=CARTESIAN_POINT ( 'NONE',  ( -18.51228436096628727, -288.1524655174525833, -196.9191759970179305 ) ) ;
#45835=CARTESIAN_POINT ( 'NONE',  ( -93.73149797201128308, -296.4088662294325900, -223.7284102769064873 ) ) ;
#45836=CARTESIAN_POINT ( 'NONE',  ( -95.57828409341681208, -290.5799529695241858, -220.1233369751405746 ) ) ;
#45837=CARTESIAN_POINT ( 'NONE',  ( 24.07674667750978514, -286.5921050256698663, -311.1086244163666947 ) ) ;
#45838=CARTESIAN_POINT ( 'NONE',  ( -78.51903429613874152, -288.1928983510649118, -331.4126532901306064 ) ) ;
#45839=CARTESIAN_POINT ( 'NONE',  ( -33.43280970683300524, -290.3418535259674513, -196.4384086568110206 ) ) ;
#45840=CARTESIAN_POINT ( 'NONE',  ( 15.30367478487448096, -288.0217514732802897, -219.2182298651522103 ) ) ;
#45841=CARTESIAN_POINT ( 'NONE',  ( -61.77904512899903011, -275.3694319698432196, -341.3230706764480260 ) ) ;
#45842=CARTESIAN_POINT ( 'NONE',  ( 37.03954081327553638, -286.1619242342672464, -286.9696773643391339 ) ) ;
#45843=CARTESIAN_POINT ( 'NONE',  ( 34.76121546066352153, -289.2844816214762318, -249.5330454387054715 ) ) ;
#45844=CARTESIAN_POINT ( 'NONE',  ( -99.18702230774165685, -287.9740693104869251, -313.0832966707152423 ) ) ;
#45845=CARTESIAN_POINT ( 'NONE',  ( -34.82649141581372731, -283.9610732389572263, -343.5656854178866411 ) ) ;
#45846=CARTESIAN_POINT ( 'NONE',  ( -107.7653581308673409, -292.8944583262457400, -243.9345845901370353 ) ) ;
#45849=CARTESIAN_POINT ( 'NONE',  ( -51.55418979226446652, -299.7920416901529279, -196.0964761880312892 ) ) ;
#45850=CARTESIAN_POINT ( 'NONE',  ( 19.80854811423548512, -280.1054384290501957, -224.6834335686284874 ) ) ;
#45851=CARTESIAN_POINT ( 'NONE',  ( 24.21203716334796496, -280.1333512500673351, -313.2112997231605505 ) ) ;
#45852=CARTESIAN_POINT ( 'NONE',  ( -8.458242663589526700, -293.8808533643207852, -341.6207406232411472 ) ) ;
#45853=CARTESIAN_POINT ( 'NONE',  ( -66.18769575042942677, -271.9091563394021591, -202.2004067812819414 ) ) ;
#45854=CARTESIAN_POINT ( 'NONE',  ( 19.39030544968409231, -274.3040769767682150, -318.5564885447232655 ) ) ;
#45855=CARTESIAN_POINT ( 'NONE',  ( -36.97638875489376886, -296.3626272252347462, -343.8658710738158675 ) ) ;
#45857=CARTESIAN_POINT ( 'NONE',  ( -112.9584881692930622, -271.2698876741405911, -259.0141153792110913 ) ) ;
#45858=CARTESIAN_POINT ( 'NONE',  ( -61.29369259105054368, -293.5987177744076462, -342.5290694644327232 ) ) ;
#45860=CARTESIAN_POINT ( 'NONE',  ( -41.64529874297971190, -293.4223034525724074, -196.8475866883864001 ) ) ;
#45862=CARTESIAN_POINT ( 'NONE',  ( 4.587837591657516256, -293.4368019563875123, -210.3447421683638368 ) ) ;
#45863=CARTESIAN_POINT ( 'NONE',  ( 202.9738562182569694, 293.9636489450776367, -54.00000000000000000 ) ) ;
#45865=CARTESIAN_POINT ( 'NONE',  ( -54.56368117419859942, -283.8520179393777880, -197.0002962274434708 ) ) ;
#45866=CARTESIAN_POINT ( 'NONE',  ( -18.22050160756444015, -294.7987543605601672, -340.8123760773518711 ) ) ;
#45868=CARTESIAN_POINT ( 'NONE',  ( -30.21489245098734244, -282.9643364679990327, -347.0305943883221289 ) ) ;
#45869=CARTESIAN_POINT ( 'NONE',  ( 30.71365686633813041, -283.0417141345947130, -237.4112278355908074 ) ) ;
#45870=CARTESIAN_POINT ( 'NONE',  ( -109.9559027117777390, -284.5413068590451644, -244.8087819912287841 ) ) ;
#45871=CARTESIAN_POINT ( 'NONE',  ( -71.02363831306909958, -289.6064229106113999, -203.5363061957213517 ) ) ;
#45872=CARTESIAN_POINT ( 'NONE',  ( 24.53363169025510260, -280.6298012115865959, -315.0392095006142199 ) ) ;
#45874=CARTESIAN_POINT ( 'NONE',  ( -39.97492824810908019, -284.7031986767851208, -196.9151542489718452 ) ) ;
#45875=CARTESIAN_POINT ( 'NONE',  ( 23.88708881022347441, -287.0899104031517481, -316.5404197950383605 ) ) ;
#45877=CARTESIAN_POINT ( 'NONE',  ( 21.98155716331697107, -295.7610955023091606, -314.2609079715049347 ) ) ;
#45878=CARTESIAN_POINT ( 'NONE',  ( -90.90296427159208292, -279.2192378610400283, -324.9310422228321045 ) ) ;
#45879=CARTESIAN_POINT ( 'NONE',  ( 36.17359573761282832, -291.7845088181169331, -286.9694433173270909 ) ) ;
#45880=CARTESIAN_POINT ( 'NONE',  ( -99.48349378287102240, -278.7486433588338741, -231.9177623336884437 ) ) ;
#45881=CARTESIAN_POINT ( 'NONE',  ( 29.47458809792505008, -293.2216069896527415, -232.0912390672972094 ) ) ;
#45882=CARTESIAN_POINT ( 'NONE',  ( -70.41347731427335077, -283.6994612225033165, -202.4231186276373364 ) ) ;
#45883=CARTESIAN_POINT ( 'NONE',  ( -106.7945155903076540, -280.1831986214629069, -298.6684857622784648 ) ) ;
#45884=CARTESIAN_POINT ( 'NONE',  ( -58.48759460446007097, -294.3911035599885508, -340.4771617555622925 ) ) ;
#45886=CARTESIAN_POINT ( 'NONE',  ( -64.78580409222807646, -295.6937435337983402, -200.5071804452682613 ) ) ;
#45890=CARTESIAN_POINT ( 'NONE',  ( 5.854930572371969788, -282.6209403198982386, -209.4850315757792316 ) ) ;
#45891=CARTESIAN_POINT ( 'NONE',  ( -106.0471977359698172, -295.7272732527312655, -295.3603277282201702 ) ) ;
#45893=CARTESIAN_POINT ( 'NONE',  ( 21.27581636871891391, -279.6952119285918457, -317.1477375740089997 ) ) ;
#45894=CARTESIAN_POINT ( 'NONE',  ( -62.75581443872281540, -296.7879991201994585, -197.9253325829729988 ) ) ;
#45895=CARTESIAN_POINT ( 'NONE',  ( 29.93705700826656013, -289.3428149920859482, -306.8981455190537986 ) ) ;
#45896=CARTESIAN_POINT ( 'NONE',  ( -73.54680841647082445, -289.3802493337931310, -333.7647253963722846 ) ) ;
#45897=CARTESIAN_POINT ( 'NONE',  ( -41.10577650072614375, -281.5240443333827329, -196.7639748144416671 ) ) ;
#45898=CARTESIAN_POINT ( 'NONE',  ( -39.21615291765332501, -299.7884859192655540, -196.3589403066428645 ) ) ;
#45900=CARTESIAN_POINT ( 'NONE',  ( -32.92386311034271529, -278.9039707970329687, -197.0971212214262778 ) ) ;
#45902=CARTESIAN_POINT ( 'NONE',  ( -111.0365049882156825, -272.6676781684890329, -247.8612628006189311 ) ) ;
#45903=CARTESIAN_POINT ( 'NONE',  ( -99.51547383516302148, -293.0301176080004097, -229.3316865498255481 ) ) ;
#45905=CARTESIAN_POINT ( 'NONE',  ( -98.19092879092313808, -290.6416895204583852, -310.8964199128417363 ) ) ;
#45907=CARTESIAN_POINT ( 'NONE',  ( -39.15794629669244387, -290.1692097272985507, -194.6052606195188162 ) ) ;
#45908=CARTESIAN_POINT ( 'NONE',  ( -37.81839704686878889, -297.7127365549954447, -197.3415298782453249 ) ) ;
#45910=CARTESIAN_POINT ( 'NONE',  ( -109.7789112840558658, -292.3788669462162488, -246.2048394368796664 ) ) ;
#45911=CARTESIAN_POINT ( 'NONE',  ( -2.659677404128715672, -288.9805209788416391, -198.2697987213421698 ) ) ;
#45912=CARTESIAN_POINT ( 'NONE',  ( 36.36884218355848475, -289.3823685569780650, -257.1548739022682071 ) ) ;
#45913=CARTESIAN_POINT ( 'NONE',  ( -36.46974125550492829, -275.0410765159518292, -345.2021562146079532 ) ) ;
#45914=CARTESIAN_POINT ( 'NONE',  ( 25.20739260042890351, -278.0213165684791079, -310.8161546156699728 ) ) ;
#45915=CARTESIAN_POINT ( 'NONE',  ( -49.90821954616613709, -289.9705764420085643, -196.9371472859167795 ) ) ;
#45916=CARTESIAN_POINT ( 'NONE',  ( -42.37208488492256464, -281.8497579877422368, -194.7634942742383544 ) ) ;
#45918=CARTESIAN_POINT ( 'NONE',  ( 33.42009158973589678, -281.1432199458240575, -288.7592941108543414 ) ) ;
#45919=CARTESIAN_POINT ( 'NONE',  ( -98.54838335215242751, -279.0136982938760752, -316.5912634602032654 ) ) ;
#45920=CARTESIAN_POINT ( 'NONE',  ( 8.956557551945696360, -281.2275180892643220, -331.3896363430529277 ) ) ;
#45921=CARTESIAN_POINT ( 'NONE',  ( -28.61584149352048811, -277.8854431548829780, -346.6816896795406819 ) ) ;
#45923=CARTESIAN_POINT ( 'NONE',  ( -7.975466246460860553, -275.9499268648332873, -199.8754128566471593 ) ) ;
#45924=CARTESIAN_POINT ( 'NONE',  ( 17.36665895637874613, -277.4090924074130839, -226.6919474004047572 ) ) ;
#45926=CARTESIAN_POINT ( 'NONE',  ( -112.0903010805062507, -298.4657364787361189, -277.1041267494484828 ) ) ;
#45928=CARTESIAN_POINT ( 'NONE',  ( -5.646392611005856210, -289.7048503962845984, -336.4643218091442805 ) ) ;
#45930=CARTESIAN_POINT ( 'NONE',  ( 9.619521467656575453, -290.1766850936639912, -330.1659808181854032 ) ) ;
#45931=CARTESIAN_POINT ( 'NONE',  ( -81.78444966438175356, -290.7773877344970970, -212.2562668699495987 ) ) ;
#45932=CARTESIAN_POINT ( 'NONE',  ( 35.88725746498300140, -287.3568517540419975, -293.9629542044079358 ) ) ;
#45934=CARTESIAN_POINT ( 'NONE',  ( -108.1164052708368928, -283.2278443668674299, -249.2703813498126522 ) ) ;
#45935=CARTESIAN_POINT ( 'NONE',  ( 13.01072771616956558, -290.2007919822636950, -324.9791207377601268 ) ) ;
#45936=CARTESIAN_POINT ( 'NONE',  ( -111.0017759286312611, -283.0609517610884041, -268.1473014485541739 ) ) ;
#45937=CARTESIAN_POINT ( 'NONE',  ( 29.41365656777395543, -282.4539380225591572, -239.4989223355257479 ) ) ;
#45938=CARTESIAN_POINT ( 'NONE',  ( 30.16151492831187397, -288.9689531535798892, -307.0255158180120247 ) ) ;
#45940=CARTESIAN_POINT ( 'NONE',  ( -70.97557322295419624, -280.0881748828659852, -205.4875467505660538 ) ) ;
#45941=CARTESIAN_POINT ( 'NONE',  ( -7.331543346083324586, -291.2319748177312704, -199.8670899874738609 ) ) ;
#45942=CARTESIAN_POINT ( 'NONE',  ( -49.32964241029981167, -286.7060347371389071, -194.4098784383886027 ) ) ;
#45943=CARTESIAN_POINT ( 'NONE',  ( -26.63587631261986033, -286.6770725324439013, -194.1176874726934329 ) ) ;
#45944=CARTESIAN_POINT ( 'NONE',  ( -76.12532518708461282, -283.7525309730459639, -332.2661121931763546 ) ) ;
#45947=CARTESIAN_POINT ( 'NONE',  ( 3.456124272871578196, -294.4544190179785801, -206.4566139546910506 ) ) ;
#45949=CARTESIAN_POINT ( 'NONE',  ( 33.98564415706008646, -292.5898197490000712, -298.0325514292105709 ) ) ;
#45951=CARTESIAN_POINT ( 'NONE',  ( -39.17563080251730412, -276.1344749856385192, -343.5734471836745456 ) ) ;
#45952=CARTESIAN_POINT ( 'NONE',  ( -73.22566530574209764, -296.9380390815718442, -202.2901947835876513 ) ) ;
#45953=CARTESIAN_POINT ( 'NONE',  ( 36.40168529197755731, -292.0375356836797778, -270.7830303976644473 ) ) ;
#45954=CARTESIAN_POINT ( 'NONE',  ( -69.68033450518434790, -295.8602609546283020, -203.7864475493039151 ) ) ;
#45955=CARTESIAN_POINT ( 'NONE',  ( -28.07132527227859597, -293.3773816730426347, -197.5008183971281710 ) ) ;
#45956=CARTESIAN_POINT ( 'NONE',  ( 15.08700164969075352, -293.8928834022941601, -219.0492086584748677 ) ) ;
#45959=CARTESIAN_POINT ( 'NONE',  ( -30.77705423703443799, -292.9691785520989811, -345.2405801251408661 ) ) ;
#45960=CARTESIAN_POINT ( 'NONE',  ( -62.92172665743409254, -299.7194103601173651, -199.8042390801840327 ) ) ;
#45961=CARTESIAN_POINT ( 'NONE',  ( 29.64511473172418476, -288.8919723450572405, -300.0872385647375609 ) ) ;
#45962=CARTESIAN_POINT ( 'NONE',  ( -72.05995984717635849, -279.4887710521282997, -337.2563642446237964 ) ) ;
#45963=CARTESIAN_POINT ( 'NONE',  ( -59.56455444407535538, -276.1286575108956072, -343.6697359188431733 ) ) ;
#45965=CARTESIAN_POINT ( 'NONE',  ( -41.17937187458611703, -273.3537660303379084, -193.5066806700255029 ) ) ;
#45966=CARTESIAN_POINT ( 'NONE',  ( 23.75290934614115912, -280.2133447556296346, -312.8906711424514242 ) ) ;
#45967=CARTESIAN_POINT ( 'NONE',  ( -5.636412383093002632, -275.0419647468469293, -339.6519192977364696 ) ) ;
#45968=CARTESIAN_POINT ( 'NONE',  ( -108.4509589499655249, -294.9929009239556876, -288.9774694734548461 ) ) ;
#45969=CARTESIAN_POINT ( 'NONE',  ( -52.77971442013231496, -275.8546258925118195, -196.9147094505850077 ) ) ;
#45970=CARTESIAN_POINT ( 'NONE',  ( -99.37135208161900835, -273.7366921289921606, -231.6801802147334683 ) ) ;
#45972=CARTESIAN_POINT ( 'NONE',  ( -110.7099506468699559, -288.7919530733773286, -253.1708118962006040 ) ) ;
#45973=CARTESIAN_POINT ( 'NONE',  ( -51.55938161639841866, -273.6986671010971008, -198.7072509640707096 ) ) ;
#45974=CARTESIAN_POINT ( 'NONE',  ( -48.74649010364381496, -299.8876356916179589, -195.8214324643442694 ) ) ;
#45975=CARTESIAN_POINT ( 'NONE',  ( -71.79703280473380289, -293.5084023905571939, -336.8048050875983677 ) ) ;
#45976=EDGE_CURVE ( 'NONE', #42078, #71834, #54199, .T. ) ;
#45977=CARTESIAN_POINT ( 'NONE',  ( -86.00800855783791121, -282.9043949343772510, -329.8232844736725724 ) ) ;
#45980=CARTESIAN_POINT ( 'NONE',  ( 30.87753300788812183, -279.1415337807155765, -239.0746429105897732 ) ) ;
#45982=CARTESIAN_POINT ( 'NONE',  ( -103.2084863280474281, -288.9106511079204438, -302.7447091870444638 ) ) ;
#45983=CARTESIAN_POINT ( 'NONE',  ( -91.66117231297106116, -281.9762546710836659, -320.9601340027639367 ) ) ;
#45984=DIRECTION ( 'NONE',  ( -1.000000000000000000, -0.000000000000000000, -0.000000000000000000 ) ) ;
#45986=CARTESIAN_POINT ( 'NONE',  ( -110.6221983677623371, -288.3462594548779521, -286.3886721057824616 ) ) ;
#45987=CARTESIAN_POINT ( 'NONE',  ( 19.52161254829543324, -276.4141706651243453, -223.4860561065499382 ) ) ;
#45988=CARTESIAN_POINT ( 'NONE',  ( -76.54144285373151035, -284.7690313170608079, -336.2358997747855369 ) ) ;
#45989=CARTESIAN_POINT ( 'NONE',  ( -10.82952857014549508, -272.4748834278478284, -199.5493953235641413 ) ) ;
#45990=CARTESIAN_POINT ( 'NONE',  ( -107.3919204476066795, -284.2798477619337518, -290.9475754062262354 ) ) ;
#45991=CARTESIAN_POINT ( 'NONE',  ( -9.750733390642082554, -278.1098333078696783, -338.5958580393216835 ) ) ;
#45992=CARTESIAN_POINT ( 'NONE',  ( 33.05602157532531749, -276.6182799060567277, -290.3258855133137786 ) ) ;
#45993=CARTESIAN_POINT ( 'NONE',  ( -37.28939128864118402, -285.0516177112871787, -345.3738304341111416 ) ) ;
#45996=CARTESIAN_POINT ( 'NONE',  ( 17.56005642389565224, -294.1273675208043983, -324.4258141224889869 ) ) ;
#45997=CARTESIAN_POINT ( 'NONE',  ( 20.78037711548910949, -288.8841746420984009, -223.5042331719720323 ) ) ;
#45999=CARTESIAN_POINT ( 'NONE',  ( -55.56934967048407970, -295.3380690714490129, -190.3538533559490702 ) ) ;
#46000=CARTESIAN_POINT ( 'NONE',  ( -109.4508417376092950, -277.1396206639161619, -296.6271607061277109 ) ) ;
#46001=CARTESIAN_POINT ( 'NONE',  ( -50.40892337213931285, -290.2878514513459436, -195.2898978625418920 ) ) ;
#46003=CARTESIAN_POINT ( 'NONE',  ( -73.91640162869806829, -287.0771190218803781, -206.3699321987036797 ) ) ;
#46004=CARTESIAN_POINT ( 'NONE',  ( -108.0785445288762077, -280.0257549532776125, -292.3103683882536643 ) ) ;
#46005=CARTESIAN_POINT ( 'NONE',  ( -12.90942351202142646, -287.7888671328199734, -197.9617384870416288 ) ) ;
#46006=CARTESIAN_POINT ( 'NONE',  ( -2.674892394259778428, -284.5939880993105362, -336.8827497383002765 ) ) ;
#46007=CARTESIAN_POINT ( 'NONE',  ( -37.12483438741440267, -277.2161514853956419, -347.3738713174889767 ) ) ;
#46008=CARTESIAN_POINT ( 'NONE',  ( -96.03517150947493519, -271.1910895208134207, -223.9380111457722080 ) ) ;
#46009=CARTESIAN_POINT ( 'NONE',  ( -113.7168233998692131, -278.5129797113544328, -260.1657597266293465 ) ) ;
#46010=CARTESIAN_POINT ( 'NONE',  ( -63.61006337088689833, -299.6273817880021397, -200.6553922133440153 ) ) ;
#46014=CARTESIAN_POINT ( 'NONE',  ( -92.74309304641960239, -295.4085103196869113, -218.6029864861167482 ) ) ;
#46016=CARTESIAN_POINT ( 'NONE',  ( -106.3243856189835839, -277.7380675174173348, -294.5848521435137286 ) ) ;
#46018=CARTESIAN_POINT ( 'NONE',  ( -85.57019588733435000, -274.6068311208042019, -210.8462382106869484 ) ) ;
#46019=CARTESIAN_POINT ( 'NONE',  ( 33.34456714679389933, -280.9946341135021157, -300.4346157586739992 ) ) ;
#46020=CARTESIAN_POINT ( 'NONE',  ( 8.626594219994279555, -290.1724069398224515, -328.3687892476896764 ) ) ;
#46021=CARTESIAN_POINT ( 'NONE',  ( -71.74396915942027420, -297.0186300703443862, -338.4727296244728336 ) ) ;
#46022=CARTESIAN_POINT ( 'NONE',  ( -106.7998472985595697, -297.3416221479740216, -302.6655218481404290 ) ) ;
#46023=CARTESIAN_POINT ( 'NONE',  ( 3.213180428380350229, -294.5981021519840510, -207.4083307871703994 ) ) ;
#46024=CARTESIAN_POINT ( 'NONE',  ( 35.55184951805858162, -279.3341532099237270, -253.4330687393945425 ) ) ;
#46025=CARTESIAN_POINT ( 'NONE',  ( -43.90188982336593426, -281.8888858114062259, -196.1595181270847092 ) ) ;
#46026=CARTESIAN_POINT ( 'NONE',  ( -102.4627073117620597, -295.1153760193253675, -234.2977207662815715 ) ) ;
#46027=CARTESIAN_POINT ( 'NONE',  ( -109.4608866148854531, -285.8390332502436308, -294.9632186082106386 ) ) ;
#46028=CARTESIAN_POINT ( 'NONE',  ( 34.87431323413013473, -286.3030342111105142, -257.4620365605622396 ) ) ;
#46029=CARTESIAN_POINT ( 'NONE',  ( 27.14702362586025686, -24.06158745657470632, -344.5372108056291154 ) ) ;
#46031=CARTESIAN_POINT ( 'NONE',  ( 33.48925405325685034, -286.4952012631553657, -299.1652243932525153 ) ) ;
#46032=CARTESIAN_POINT ( 'NONE',  ( 35.47262882870926148, -287.2996604936064386, -276.4873326521638432 ) ) ;
#46034=CARTESIAN_POINT ( 'NONE',  ( -109.9276649085463475, -285.3186601792354509, -295.1153141182892341 ) ) ;
#46035=CARTESIAN_POINT ( 'NONE',  ( 25.39590465244069506, -276.3989775775290241, -307.7252777231987579 ) ) ;
#46036=CARTESIAN_POINT ( 'NONE',  ( -53.31147274504701272, -290.7724350610319561, -195.2971156415540293 ) ) ;
#46037=CARTESIAN_POINT ( 'NONE',  ( 21.53732274481225772, -282.8704325085367373, -319.8239671978680576 ) ) ;
#46039=CARTESIAN_POINT ( 'NONE',  ( -106.7961564113329587, -280.4813262075144280, -238.6302487405615693 ) ) ;
#46040=CARTESIAN_POINT ( 'NONE',  ( 35.30632078384844874, -281.5624724457769048, -244.7459096834286925 ) ) ;
#46041=CARTESIAN_POINT ( 'NONE',  ( 30.89617123739170168, -279.2666405000204009, -285.9686137636504668 ) ) ;
#46042=CARTESIAN_POINT ( 'NONE',  ( 168.7673636147504510, 232.2389198171512135, -192.7723113846432739 ) ) ;
#46044=CARTESIAN_POINT ( 'NONE',  ( 25.53837903002381893, -278.1013100879092121, -311.0291679278843162 ) ) ;
#46045=CARTESIAN_POINT ( 'NONE',  ( -108.3824614259837631, -261.6036692187849440, -317.2910301733635947 ) ) ;
#46046=CARTESIAN_POINT ( 'NONE',  ( 5.895960732329615261, -278.6617934428740568, -209.5141666752244021 ) ) ;
#46047=CARTESIAN_POINT ( 'NONE',  ( -108.5744972866913258, -296.1171096757910846, -253.9360981180980161 ) ) ;
#46048=CARTESIAN_POINT ( 'NONE',  ( 36.30895030370150067, -293.3413636572570340, -292.7925800508041903 ) ) ;
#46049=DIRECTION ( 'NONE',  ( 0.000000000000000000, 0.000000000000000000, 1.000000000000000000 ) ) ;
#46050=CARTESIAN_POINT ( 'NONE',  ( -30.53152898055697406, -296.7105726661367271, -193.9519552065307835 ) ) ;
#46051=CARTESIAN_POINT ( 'NONE',  ( -107.7211338833747760, -288.6588367221238514, -292.7378521487297576 ) ) ;
#46052=CARTESIAN_POINT ( 'NONE',  ( -80.86004922154192798, -297.5103707697078903, -330.5027738455837039 ) ) ;
#46053=CARTESIAN_POINT ( 'NONE',  ( -30.50195517935300771, -287.4554877727456415, -197.1357917279403864 ) ) ;
#46054=CARTESIAN_POINT ( 'NONE',  ( 38.12814325710726138, -294.6704202427430914, -284.4722503976491339 ) ) ;
#46055=CARTESIAN_POINT ( 'NONE',  ( -109.0386762002837457, -284.8592535442434155, -284.4157280420699294 ) ) ;
#46056=CARTESIAN_POINT ( 'NONE',  ( -95.26074806815006468, -296.0285323846819097, -220.1482243354519994 ) ) ;
#46057=CARTESIAN_POINT ( 'NONE',  ( -61.64721639579236268, -292.5471606104630382, -197.4119989845897862 ) ) ;
#46058=CARTESIAN_POINT ( 'NONE',  ( -77.14280097261693925, -292.0264723446757102, -204.4559232188687474 ) ) ;
#46059=CARTESIAN_POINT ( 'NONE',  ( -58.68710308437942302, -289.5025650551257286, -340.2234750382236825 ) ) ;
#46062=CARTESIAN_POINT ( 'NONE',  ( -54.34142713924888568, -299.6964516281937563, -196.5280985446813702 ) ) ;
#46063=CARTESIAN_POINT ( 'NONE',  ( -69.94873143957963180, -272.4271628616909879, -201.0301858255633931 ) ) ;
#46064=CARTESIAN_POINT ( 'NONE',  ( 3.511569450750162247, -281.5468631406942563, -331.2041848219550388 ) ) ;
#46066=CARTESIAN_POINT ( 'NONE',  ( -31.46123135671274085, -276.4875695285002166, -347.1271073884383895 ) ) ;
#46067=CARTESIAN_POINT ( 'NONE',  ( -35.77790516194551884, -296.5519523500449282, -196.6681930200876707 ) ) ;
#46068=CARTESIAN_POINT ( 'NONE',  ( -109.9683794781587665, -280.2131890049852245, -285.7309237709808940 ) ) ;
#46069=CARTESIAN_POINT ( 'NONE',  ( 31.41323946870123862, -274.0620890358339921, -298.4910705554410129 ) ) ;
#46070=CARTESIAN_POINT ( 'NONE',  ( -109.5298882069641877, -297.5822606652396303, -283.6970119927557334 ) ) ;
#46071=CARTESIAN_POINT ( 'NONE',  ( -109.3633214737600099, -273.6715681474125290, -256.8120217745229183 ) ) ;
#46072=CARTESIAN_POINT ( 'NONE',  ( -94.97949383970086501, -298.8332832250812885, -220.4393361434963197 ) ) ;
#46073=CARTESIAN_POINT ( 'NONE',  ( -21.67168307186484810, -272.2721735945495993, -196.6531986982309945 ) ) ;
#46074=CARTESIAN_POINT ( 'NONE',  ( 34.04755592211761694, -293.9955752367482660, -254.5721886120804811 ) ) ;
#46075=CARTESIAN_POINT ( 'NONE',  ( -47.05441299881726280, -290.5010844398804011, -197.4156717577427571 ) ) ;
#46076=CARTESIAN_POINT ( 'NONE',  ( 115.2448031289451222, -299.5541904835127980, -195.3611179825600175 ) ) ;
#46077=CARTESIAN_POINT ( 'NONE',  ( -75.30037756694086681, -278.0365520000658535, -337.2839519808595128 ) ) ;
#46078=CARTESIAN_POINT ( 'NONE',  ( -47.27982467328074989, -298.2558154095355007, -197.9681949448096248 ) ) ;
#46079=CARTESIAN_POINT ( 'NONE',  ( 6.627811149647447664, -281.1532837015721498, -333.0356375875309141 ) ) ;
#46080=CARTESIAN_POINT ( 'NONE',  ( -58.31476465329029679, -297.3226295194288014, -342.5967924246133407 ) ) ;
#46082=CARTESIAN_POINT ( 'NONE',  ( -59.00567902545960663, -282.5367725711949447, -340.2948043582983360 ) ) ;
#46084=CARTESIAN_POINT ( 'NONE',  ( -69.70443733715549683, -281.4769820109128204, -338.2183035407334728 ) ) ;
#46085=CARTESIAN_POINT ( 'NONE',  ( 34.08544686764336262, -273.8950887982017548, -252.6541252724424567 ) ) ;
#46086=CARTESIAN_POINT ( 'NONE',  ( 31.97045156365387797, -283.1769049838175647, -241.5774200847378665 ) ) ;
#46089=CARTESIAN_POINT ( 'NONE',  ( 0.8126862128197108737, -272.9520237599154484, -204.3862805540542809 ) ) ;
#46091=CARTESIAN_POINT ( 'NONE',  ( -112.5441497201053522, -280.5723370762114541, -268.7983991541806859 ) ) ;
#46094=CARTESIAN_POINT ( 'NONE',  ( 32.51853913141793129, -289.0978927903359477, -241.4345894216269244 ) ) ;
#46096=CARTESIAN_POINT ( 'NONE',  ( -97.83258073832952562, -289.1567327142652175, -226.0017343830446634 ) ) ;
#46098=CARTESIAN_POINT ( 'NONE',  ( -82.61674104850737876, -294.4812464764269180, -328.1953066264362064 ) ) ;
#46099=CARTESIAN_POINT ( 'NONE',  ( -98.37777008258306921, -288.1125832734024357, -312.6382074147545040 ) ) ;
#46100=CARTESIAN_POINT ( 'NONE',  ( 175.8323451578035872, 256.8656992060370499, -165.6361338323774817 ) ) ;
#46101=CARTESIAN_POINT ( 'NONE',  ( -110.8499041012236432, -294.3600576685423675, -285.3095547068453470 ) ) ;
#46102=CARTESIAN_POINT ( 'NONE',  ( 36.46880007786586475, -286.2765498069288128, -289.7187473239187057 ) ) ;
#46103=CARTESIAN_POINT ( 'NONE',  ( 22.75321873640402970, -282.5603315451539856, -227.5237377775503376 ) ) ;
#46104=CARTESIAN_POINT ( 'NONE',  ( -71.30618411785034993, -281.7343057551539118, -338.3345528254463375 ) ) ;
#46105=CARTESIAN_POINT ( 'NONE',  ( -109.4191042533716001, -290.3984972085565346, -282.0090036074795989 ) ) ;
#46106=CARTESIAN_POINT ( 'NONE',  ( 36.10685697529019933, -282.9179161881680216, -265.8131101515400019 ) ) ;
#46107=CARTESIAN_POINT ( 'NONE',  ( 35.72770680629005113, -282.4032864712268633, -274.0303817727408955 ) ) ;
#46109=CARTESIAN_POINT ( 'NONE',  ( 6.987731734248881388, -290.4323270380440363, -331.3623997911580545 ) ) ;
#46110=CARTESIAN_POINT ( 'NONE',  ( -35.47404145034176537, -298.2416097282461465, -193.3610667654473048 ) ) ;
#46112=CARTESIAN_POINT ( 'NONE',  ( 36.49346288353235934, -275.8267837741274775, -292.2564064448038152 ) ) ;
#46113=CARTESIAN_POINT ( 'NONE',  ( -17.00823401897600107, -294.2957439519510103, -198.4853655749896859 ) ) ;
#46115=CARTESIAN_POINT ( 'NONE',  ( -54.49178911615187815, -288.3376638359845856, -195.3683826091709363 ) ) ;
#46116=CARTESIAN_POINT ( 'NONE',  ( 34.72823422483048006, -273.8269462194310790, -291.7595326021432243 ) ) ;
#46118=CARTESIAN_POINT ( 'NONE',  ( -59.89169825058520047, -296.1647467918778034, -197.5192424894375733 ) ) ;
#46119=CARTESIAN_POINT ( 'NONE',  ( -109.1238519256437485, -291.9286130720112169, -287.5006366707467578 ) ) ;
#46120=CARTESIAN_POINT ( 'NONE',  ( -6.478410830761558437, -273.8171486289658674, -204.0938557613360160 ) ) ;
#46121=CARTESIAN_POINT ( 'NONE',  ( -88.42502221032009402, -292.8408530846274402, -217.1755890785530312 ) ) ;
#46122=CARTESIAN_POINT ( 'NONE',  ( -95.30795483998606699, -292.1215232765439396, -225.6026353951364172 ) ) ;
#46123=CARTESIAN_POINT ( 'NONE',  ( -109.9695987778565893, -286.1268425734511993, -284.6146211767700152 ) ) ;
#46124=CARTESIAN_POINT ( 'NONE',  ( -113.8003228525353308, -291.9663440890844299, -271.2402333106921333 ) ) ;
#46125=CARTESIAN_POINT ( 'NONE',  ( -37.80893251760928564, -293.3615821891834230, -193.8556935414138991 ) ) ;
#46126=CARTESIAN_POINT ( 'NONE',  ( 6.061235767508152961, -294.2782533263938376, -329.1198124285405129 ) ) ;
#46127=CARTESIAN_POINT ( 'NONE',  ( 33.29128194310850120, -289.8791274019168327, -295.5798112708931171 ) ) ;
#46128=CARTESIAN_POINT ( 'NONE',  ( 29.76294148372031501, -282.2099935017037637, -308.2317696016779678 ) ) ;
#46129=CARTESIAN_POINT ( 'NONE',  ( 6.960833408849198989, -296.6824680553923486, -194.8154681501593757 ) ) ;
#46130=CARTESIAN_POINT ( 'NONE',  ( -60.50789903976123441, -285.5932377349557214, -196.8730753921845462 ) ) ;
#46131=CARTESIAN_POINT ( 'NONE',  ( 37.34497197834174642, -277.5478703728319942, -271.5873799267992013 ) ) ;
#46132=CARTESIAN_POINT ( 'NONE',  ( -87.20981319408446097, -282.5603489076043502, -324.2851145895770628 ) ) ;
#46133=CARTESIAN_POINT ( 'NONE',  ( 20.56273307833539477, -284.8945380617355454, -222.6948063175437369 ) ) ;
#46134=CARTESIAN_POINT ( 'NONE',  ( -77.18580578217274990, -275.7193696026913585, -334.8639504470550037 ) ) ;
#46136=CARTESIAN_POINT ( 'NONE',  ( -4.805385398037338440, -282.1192531753392814, -335.7780627725132376 ) ) ;
#46137=CARTESIAN_POINT ( 'NONE',  ( -35.36175165022358868, -281.2815239598371022, -193.7707118762414780 ) ) ;
#46138=CARTESIAN_POINT ( 'NONE',  ( 37.15140899565254529, -286.3782900832634937, -251.8247508377432951 ) ) ;
#46139=CARTESIAN_POINT ( 'NONE',  ( 8.878219529811792299, -296.1687571370302408, -328.2343802652337672 ) ) ;
#46140=CARTESIAN_POINT ( 'NONE',  ( 38.58511446579264970, -277.2337496475062721, -276.8077635946577857 ) ) ;
#46141=CARTESIAN_POINT ( 'NONE',  ( 39.21410212106193427, -276.8772512868949889, -271.1497358663002615 ) ) ;
#46142=CARTESIAN_POINT ( 'NONE',  ( -95.27431517163964259, -277.7605854553406175, -314.7774676608826212 ) ) ;
#46143=CARTESIAN_POINT ( 'NONE',  ( -42.00746948066868924, -299.9933605363592051, -195.6733745165925029 ) ) ;
#46144=CARTESIAN_POINT ( 'NONE',  ( 32.17915235270469054, -285.9150837590440801, -298.1933438291356424 ) ) ;
#46145=CARTESIAN_POINT ( 'NONE',  ( -111.5429616737715293, -292.3713940528133435, -253.0229172766923398 ) ) ;
#46146=CARTESIAN_POINT ( 'NONE',  ( -71.08526816811954063, -294.4287426400462095, -335.4566322670959266 ) ) ;
#46148=CARTESIAN_POINT ( 'NONE',  ( 29.87687044034836958, -292.8344390153208110, -241.7054125770505095 ) ) ;
#46150=CARTESIAN_POINT ( 'NONE',  ( 0.5784681257780236452, -289.6390423541757855, -337.0811170808499355 ) ) ;
#46151=CARTESIAN_POINT ( 'NONE',  ( -83.50852691119169435, -280.0512935461091502, -213.6165257675015141 ) ) ;
#46152=CARTESIAN_POINT ( 'NONE',  ( -106.8918469178613577, -295.0572427316778317, -302.6762783627173690 ) ) ;
#46153=CARTESIAN_POINT ( 'NONE',  ( 38.87313931373427067, -288.0754790186344394, -260.1331643561269971 ) ) ;
#46154=CARTESIAN_POINT ( 'NONE',  ( 24.68371495242304547, -287.2796616143220376, -224.7695378862669600 ) ) ;
#46155=CARTESIAN_POINT ( 'NONE',  ( -108.7398411792730144, -284.6827468380653272, -285.7303862886270167 ) ) ;
#46156=CARTESIAN_POINT ( 'NONE',  ( -22.58273187487147382, -108.0340517555389539, -362.5798773164099202 ) ) ;
#46157=CARTESIAN_POINT ( 'NONE',  ( -96.21878309525817485, -238.5862671180402970, -340.1699584742321463 ) ) ;
#46158=CARTESIAN_POINT ( 'NONE',  ( -94.19091026945986300, -238.5270531376727092, -338.5184284098635885 ) ) ;
#46160=CARTESIAN_POINT ( 'NONE',  ( -66.87720454847166707, -276.6465701445121113, -337.2958302476669132 ) ) ;
#46161=CARTESIAN_POINT ( 'NONE',  ( -71.81163762643308246, -276.4393281188836227, -335.0749653636798939 ) ) ;
#46162=CARTESIAN_POINT ( 'NONE',  ( -29.06155764960093535, -297.6608735929614227, -193.4233259703201213 ) ) ;
#46163=CARTESIAN_POINT ( 'NONE',  ( -61.49889831844556909, -183.5886210442853326, -359.5431637745206785 ) ) ;
#46164=CARTESIAN_POINT ( 'NONE',  ( -35.73874141804396487, -275.7173027604336539, -346.8642145531776464 ) ) ;
#46165=CARTESIAN_POINT ( 'NONE',  ( -72.38287194409117831, -290.0216038275953565, -334.4712164034065154 ) ) ;
#46166=CARTESIAN_POINT ( 'NONE',  ( -46.12159095762173422, -298.7463025151313332, -194.0258552446377394 ) ) ;
#46167=CARTESIAN_POINT ( 'NONE',  ( -34.05652319490675950, -298.5845947084019372, -193.4223898508425918 ) ) ;
#46168=CARTESIAN_POINT ( 'NONE',  ( 12.35642799949807191, -294.5037644111103532, -323.9009182221352603 ) ) ;
#46170=CARTESIAN_POINT ( 'NONE',  ( -38.49793388571393393, -278.9866928105701049, -345.9122749908211176 ) ) ;
#46171=CARTESIAN_POINT ( 'NONE',  ( -47.25464769423852118, -282.6825557864519851, -346.6583025549425088 ) ) ;
#46172=CARTESIAN_POINT ( 'NONE',  ( -109.7954839753122229, -279.4851534149324266, -281.5269265103479484 ) ) ;
#46173=CARTESIAN_POINT ( 'NONE',  ( -42.71188665963277487, -278.8791768597490091, -346.1577875048786836 ) ) ;
#46174=CARTESIAN_POINT ( 'NONE',  ( -47.33494322860493497, -296.4975451618913098, -197.4019512077545926 ) ) ;
#46176=CARTESIAN_POINT ( 'NONE',  ( -108.7643344056090626, -278.5197271859262287, -285.4544051458017861 ) ) ;
#46177=CARTESIAN_POINT ( 'NONE',  ( -38.36553560907224636, -274.8424518016485081, -193.5294150068752401 ) ) ;
#46178=CARTESIAN_POINT ( 'NONE',  ( 9.910132642451632279, -287.1018647103783792, -330.5996140805041819 ) ) ;
#46179=CARTESIAN_POINT ( 'NONE',  ( -68.04912357407837931, -275.6491723184861939, -201.9215521663130630 ) ) ;
#46180=CARTESIAN_POINT ( 'NONE',  ( 39.11759607059777011, -274.1372459535500639, -271.1835561986710559 ) ) ;
#46182=CARTESIAN_POINT ( 'NONE',  ( -74.80735642719723444, -288.7618933278195641, -333.2163215201099433 ) ) ;
#46183=CARTESIAN_POINT ( 'NONE',  ( -69.74232232338688675, -284.9852853829084438, -200.6078844102750054 ) ) ;
#46185=CARTESIAN_POINT ( 'NONE',  ( -15.85949873780902486, -281.0102811206787692, -341.1882952171815191 ) ) ;
#46186=CARTESIAN_POINT ( 'NONE',  ( 22.27874692674471291, -280.7257744381483917, -313.5194134312836240 ) ) ;
#46187=CARTESIAN_POINT ( 'NONE',  ( -60.40195178713290147, -283.8306126534583314, -199.5830211613755978 ) ) ;
#46188=CARTESIAN_POINT ( 'NONE',  ( -32.53978009027839136, -290.9919073492675352, -345.2577204400344613 ) ) ;
#46189=CARTESIAN_POINT ( 'NONE',  ( 19.13184210540476826, -282.0957184221804255, -223.4601759565237842 ) ) ;
#46190=CARTESIAN_POINT ( 'NONE',  ( 201.7240241153841396, 293.7293971333333502, -83.18315278848760386 ) ) ;
#46191=CARTESIAN_POINT ( 'NONE',  ( -16.38165683845463505, -281.1856673722065807, -343.6764346845136515 ) ) ;
#46192=CARTESIAN_POINT ( 'NONE',  ( 12.09710782999317935, -296.3652147601297884, -326.8286230029559079 ) ) ;
#46193=CARTESIAN_POINT ( 'NONE',  ( -95.12050561012156891, -277.4667845066937275, -220.9895076386954429 ) ) ;
#46194=CARTESIAN_POINT ( 'NONE',  ( -33.13525807552652935, -284.9994731475740650, -345.4228192937957260 ) ) ;
#46196=CARTESIAN_POINT ( 'NONE',  ( -9.073077035165718840, -294.3391085262769593, -200.2883048003837132 ) ) ;
#46197=CARTESIAN_POINT ( 'NONE',  ( -9.262593979212509154, -274.6849535548248582, -339.9204659320925543 ) ) ;
#46198=CARTESIAN_POINT ( 'NONE',  ( 37.56451522790833053, -286.5340600598635206, -253.1790870622292573 ) ) ;
#46199=CARTESIAN_POINT ( 'NONE',  ( -108.1572578066967196, -289.2244274860439646, -249.5413717850366311 ) ) ;
#46201=CARTESIAN_POINT ( 'NONE',  ( -32.40404411641769400, -275.6735592464879687, -343.7385183722637407 ) ) ;
#46202=CARTESIAN_POINT ( 'NONE',  ( -56.13857124124354669, -293.4362809411676949, -342.2304293144740654 ) ) ;
#46203=CARTESIAN_POINT ( 'NONE',  ( -80.68493099996972262, -290.9688177891488863, -329.7759957522601439 ) ) ;
#46204=DIRECTION ( 'NONE',  ( -0.8510748438184358999, -0.5250018354872690862, -0.006684530980050039546 ) ) ;
#46206=CARTESIAN_POINT ( 'NONE',  ( 30.29343671947234640, -291.5708014247982760, -234.9174954872486296 ) ) ;
#46207=CARTESIAN_POINT ( 'NONE',  ( -37.30066544658166805, -287.6527672658560277, -196.5485513742615069 ) ) ;
#46208=CARTESIAN_POINT ( 'NONE',  ( -38.92187258964147389, -287.3115867626428894, -346.3313560473806660 ) ) ;
#46210=CARTESIAN_POINT ( 'NONE',  ( 35.57749773118361958, -288.8429135475420821, -260.0817373403651231 ) ) ;
#46212=CARTESIAN_POINT ( 'NONE',  ( 35.61377461783489906, -288.4355912920238438, -276.4846964328231138 ) ) ;
#46213=CARTESIAN_POINT ( 'NONE',  ( -70.07020273953243361, -297.4609553166690716, -338.2520569839953737 ) ) ;
#46215=CARTESIAN_POINT ( 'NONE',  ( 32.34439647979730381, -288.3470231621623157, -238.4237866358001838 ) ) ;
#46216=CARTESIAN_POINT ( 'NONE',  ( -68.44538412627868240, -275.5374287157678168, -339.2365295896872794 ) ) ;
#46217=CARTESIAN_POINT ( 'NONE',  ( -65.08348895615139895, -277.7380180020664397, -342.2236364944200773 ) ) ;
#46218=CARTESIAN_POINT ( 'NONE',  ( 12.98155465945337461, -280.3995669858319957, -212.1089564859341863 ) ) ;
#46219=CARTESIAN_POINT ( 'NONE',  ( -33.73733337003511679, -300.0773764445695519, -195.7150858637083957 ) ) ;
#46221=CARTESIAN_POINT ( 'NONE',  ( -95.66159568953476366, -283.2013669031691734, -223.1836902519604848 ) ) ;
#46223=CARTESIAN_POINT ( 'NONE',  ( -106.6593017720220047, -277.0423655071184044, -243.6478120152501674 ) ) ;
#46224=CARTESIAN_POINT ( 'NONE',  ( 35.59721309109747978, -279.7768593533121475, -287.8776510799567632 ) ) ;
#46226=CARTESIAN_POINT ( 'NONE',  ( -8.167785558938920332, -275.1568502994144865, -340.8847784349513290 ) ) ;
#46227=CARTESIAN_POINT ( 'NONE',  ( -110.7885212765913394, -297.9857752888462983, -276.9810065763996363 ) ) ;
#46228=CARTESIAN_POINT ( 'NONE',  ( -19.00568053621997322, -281.7419514220003407, -344.8825090160722766 ) ) ;
#46229=CARTESIAN_POINT ( 'NONE',  ( -108.0660035123709690, -297.7442958759102112, -251.3001007439489172 ) ) ;
#46230=CARTESIAN_POINT ( 'NONE',  ( -35.85699853961065031, -299.3855416260925040, -193.8539410945947452 ) ) ;
#46231=CARTESIAN_POINT ( 'NONE',  ( -34.03547643599088701, -273.7615982031505268, -197.4148612470219746 ) ) ;
#46232=CARTESIAN_POINT ( 'NONE',  ( 37.28268231497051488, -295.4496335698748908, -262.3640191090117355 ) ) ;
#46233=CARTESIAN_POINT ( 'NONE',  ( 38.67532562284709030, -287.8762676522165407, -282.9495830547723472 ) ) ;
#46234=CARTESIAN_POINT ( 'NONE',  ( -104.8773269271692641, -277.0775491069227883, -236.3587750604658879 ) ) ;
#46235=CARTESIAN_POINT ( 'NONE',  ( -96.57750882963703987, -291.0471746808080979, -221.1460381611533705 ) ) ;
#46236=CARTESIAN_POINT ( 'NONE',  ( 20.53605821534826603, -287.2410821642815790, -315.2542774257673273 ) ) ;
#46237=CARTESIAN_POINT ( 'NONE',  ( -2.949655718037113239, -290.5064174255074363, -203.6969813962691944 ) ) ;
#46239=CARTESIAN_POINT ( 'NONE',  ( -114.4693268140674434, -273.6886850827510216, -284.2063049943780015 ) ) ;
#46240=CARTESIAN_POINT ( 'NONE',  ( 32.37044432901250701, -287.3513885459868789, -292.3973599499830129 ) ) ;
#46242=CARTESIAN_POINT ( 'NONE',  ( -110.8791176002514902, -285.2156470433626509, -292.4310086095234738 ) ) ;
#46243=CARTESIAN_POINT ( 'NONE',  ( 39.00173524470162789, -292.7177781905338634, -278.8806994840650191 ) ) ;
#46244=CARTESIAN_POINT ( 'NONE',  ( 36.50458824150194204, -282.6146664768839400, -250.3108789574148716 ) ) ;
#46245=CARTESIAN_POINT ( 'NONE',  ( -21.39028187699264194, -282.6752953878387302, -341.6490221656364952 ) ) ;
#46246=CARTESIAN_POINT ( 'NONE',  ( -102.3163945606061134, -297.0937311082029169, -229.0417631545857375 ) ) ;
#46247=CARTESIAN_POINT ( 'NONE',  ( -48.96986659486070437, -275.2162387408656627, -197.7421859769735022 ) ) ;
#46248=CARTESIAN_POINT ( 'NONE',  ( -60.75140536285802995, -289.7671641781465155, -199.4278911509432533 ) ) ;
#46249=CARTESIAN_POINT ( 'NONE',  ( -29.93461739507998942, -272.9429115437400810, -197.3387540790971570 ) ) ;
#46252=CARTESIAN_POINT ( 'NONE',  ( -8.966684677925307767, -288.3463165669435853, -201.5274890656250193 ) ) ;
#46253=CARTESIAN_POINT ( 'NONE',  ( -11.14980158982232794, -295.7984535440176046, -342.4971213971670636 ) ) ;
#46254=CARTESIAN_POINT ( 'NONE',  ( -108.7662776926124479, -285.4094440141853397, -254.7327277577390987 ) ) ;
#46255=CARTESIAN_POINT ( 'NONE',  ( 39.08426611691788111, -274.5137425103191617, -262.6160379171742534 ) ) ;
#46256=CARTESIAN_POINT ( 'NONE',  ( -16.66200996197529349, -292.9639359549618121, -196.2958548632652764 ) ) ;
#46257=CARTESIAN_POINT ( 'NONE',  ( 19.37805501915875084, -284.9995547954317203, -220.0524283685683997 ) ) ;
#46258=CARTESIAN_POINT ( 'NONE',  ( 23.15769014751301214, -294.5223369966837481, -317.9802518562189562 ) ) ;
#46259=CARTESIAN_POINT ( 'NONE',  ( -110.2670399689955190, -290.9463977190860078, -265.7385080512584636 ) ) ;
#46262=CARTESIAN_POINT ( 'NONE',  ( -30.06861358815306318, -125.2304951651611020, -360.6161781973373763 ) ) ;
#46263=CARTESIAN_POINT ( 'NONE',  ( -65.63840940208109487, -287.2088798734749844, -199.4809900978910946 ) ) ;
#46264=CARTESIAN_POINT ( 'NONE',  ( -72.02372285203398405, -271.1237833571632905, -198.2697987213421698 ) ) ;
#46266=CARTESIAN_POINT ( 'NONE',  ( -108.0629762411944768, -283.2179300521741538, -289.7146892801354170 ) ) ;
#46267=CARTESIAN_POINT ( 'NONE',  ( -82.53729739451570424, -277.3177300720651033, -332.6756610617824208 ) ) ;
#46268=CARTESIAN_POINT ( 'NONE',  ( 36.51702530783049383, -283.7072261746205299, -282.3992700271738272 ) ) ;
#46269=CARTESIAN_POINT ( 'NONE',  ( -54.04194081808444139, -170.5257408106840558, -363.2615279374122679 ) ) ;
#46270=CARTESIAN_POINT ( 'NONE',  ( -66.36934788348081327, -281.9995673580031053, -341.0575990416611489 ) ) ;
#46271=CARTESIAN_POINT ( 'NONE',  ( 35.31704978269277007, -285.3508884591338983, -253.2016229601303792 ) ) ;
#46272=CARTESIAN_POINT ( 'NONE',  ( -101.6827884767155012, -274.9444500212786124, -230.3544956636292511 ) ) ;
#46273=CARTESIAN_POINT ( 'NONE',  ( -58.42000539663133907, -295.8244719080564664, -340.3160569684570191 ) ) ;
#46274=ORIENTED_EDGE ( 'NONE', *, *, #67056, .F. ) ;
#46275=CARTESIAN_POINT ( 'NONE',  ( -47.04309644520665756, -290.6111649840099176, -197.5110913060013331 ) ) ;
#46276=CARTESIAN_POINT ( 'NONE',  ( -113.6640153480350932, -279.0806679341160361, -280.1747311104796268 ) ) ;
#46277=CARTESIAN_POINT ( 'NONE',  ( 35.60193609077818877, -275.6042791801405087, -274.3126303681194713 ) ) ;
#46278=CARTESIAN_POINT ( 'NONE',  ( 30.26405250746054421, -274.9436141718023805, -306.6803198339683831 ) ) ;
#46280=CARTESIAN_POINT ( 'NONE',  ( -33.50494521547745563, -272.1002650189423662, -195.4466888876256974 ) ) ;
#46282=CARTESIAN_POINT ( 'NONE',  ( -11.24128429275440233, -296.1439987217785301, -342.2321231324961559 ) ) ;
#46285=CARTESIAN_POINT ( 'NONE',  ( -110.6187084289727949, -285.6603267123361434, -268.1917569814370381 ) ) ;
#46286=CARTESIAN_POINT ( 'NONE',  ( -24.68006851802043400, -284.6530082800641139, -345.3388667412988866 ) ) ;
#46287=CARTESIAN_POINT ( 'NONE',  ( -78.44077709836832923, -282.9703452669656372, -330.8157169816710166 ) ) ;
#46288=CARTESIAN_POINT ( 'NONE',  ( 10.16362670252486566, -274.7839992825527702, -326.8384084257006066 ) ) ;
#46289=CARTESIAN_POINT ( 'NONE',  ( 26.63537936562969222, -283.9223222138413121, -308.1164186136542753 ) ) ;
#46290=CARTESIAN_POINT ( 'NONE',  ( -67.10022423793390089, -275.9293967296944174, -337.7787565998945070 ) ) ;
#46291=CARTESIAN_POINT ( 'NONE',  ( 20.27390275724414437, -277.2687251126907881, -315.7097886556133517 ) ) ;
#46293=CARTESIAN_POINT ( 'NONE',  ( -94.84774534786933486, -280.0468785297908880, -219.3982532288467837 ) ) ;
#46294=CARTESIAN_POINT ( 'NONE',  ( -62.03382016110933250, -280.2320118665113569, -197.4363751072278887 ) ) ;
#46297=CARTESIAN_POINT ( 'NONE',  ( 38.37123740727610510, -289.4630672738114754, -274.3341554334433567 ) ) ;
#46298=CARTESIAN_POINT ( 'NONE',  ( -108.1284044367303778, -295.5051595200919223, -288.8997070272046699 ) ) ;
#46299=CARTESIAN_POINT ( 'NONE',  ( -71.86814614747392227, -288.8451493913223089, -339.0723784303086745 ) ) ;
#46301=CARTESIAN_POINT ( 'NONE',  ( 3.018101175348274268, -284.8421288870412127, -208.3203213164763667 ) ) ;
#46302=CARTESIAN_POINT ( 'NONE',  ( -9.251810149712797582, -285.0014304847313724, -202.3303471054953206 ) ) ;
#46303=CARTESIAN_POINT ( 'NONE',  ( -103.7645765641147051, -288.3556749469547071, -303.0103981713608619 ) ) ;
#46304=CARTESIAN_POINT ( 'NONE',  ( -91.82623210097115418, -286.4583933362018229, -221.1074983045434976 ) ) ;
#46305=CARTESIAN_POINT ( 'NONE',  ( -48.22949183385324545, -275.1904010738356874, -344.6191174926257759 ) ) ;
#46306=CARTESIAN_POINT ( 'NONE',  ( 11.88335065627740761, -286.7811178905666907, -328.5275583819951635 ) ) ;
#46307=CARTESIAN_POINT ( 'NONE',  ( 20.53024547613670237, -288.8942117152043352, -222.6553681751702243 ) ) ;
#46308=CARTESIAN_POINT ( 'NONE',  ( 21.82814721845769412, -286.1869833289202347, -316.7386852402980821 ) ) ;
#46309=CARTESIAN_POINT ( 'NONE',  ( 14.09845758317911013, -283.2496735033903974, -322.5604379622570264 ) ) ;
#46310=CARTESIAN_POINT ( 'NONE',  ( 19.21079913231912073, -290.2386823653113197, -319.8966076060448245 ) ) ;
#46313=CARTESIAN_POINT ( 'NONE',  ( -72.63029377766190464, -299.5091890795721383, -203.4899686540603057 ) ) ;
#46315=CARTESIAN_POINT ( 'NONE',  ( 37.70371272009514740, -279.5648804318485077, -271.3652785254038804 ) ) ;
#46316=CARTESIAN_POINT ( 'NONE',  ( -11.19855715296629661, -291.5813785442620656, -198.0508182402863326 ) ) ;
#46317=CARTESIAN_POINT ( 'NONE',  ( -111.1741663943203662, -294.9737602023050158, -268.6947196850270529 ) ) ;
#46318=CARTESIAN_POINT ( 'NONE',  ( 32.45017119036801745, -279.9314194999859069, -247.1715353946632092 ) ) ;
#46319=CARTESIAN_POINT ( 'NONE',  ( 12.52903630444056304, -272.8329343424976514, -215.0266566773978241 ) ) ;
#46320=CARTESIAN_POINT ( 'NONE',  ( -95.98780272191407903, -297.2490271468528817, -314.6749368759372487 ) ) ;
#46322=CARTESIAN_POINT ( 'NONE',  ( 7.501621120913360308, -297.0838201114648882, -194.0657894636586036 ) ) ;
#46323=CARTESIAN_POINT ( 'NONE',  ( 20.58048956254331685, -292.4638758398115215, -319.5443870633923211 ) ) ;
#46325=CARTESIAN_POINT ( 'NONE',  ( -70.50235700857385268, -293.0313014536339438, -204.6667821989525464 ) ) ;
#46326=CARTESIAN_POINT ( 'NONE',  ( 129.9467878515196162, -299.5541904835127980, -195.3611179825600175 ) ) ;
#46327=CARTESIAN_POINT ( 'NONE',  ( 34.48485135541626079, -294.5381067991047530, -284.2732791867372271 ) ) ;
#46328=FACE_BOUND ( 'NONE', #79109, .T. ) ;
#46329=CARTESIAN_POINT ( 'NONE',  ( -41.50405241988473648, -281.1243016670110819, -345.6524856356463715 ) ) ;
#46330=CARTESIAN_POINT ( 'NONE',  ( -45.09073446984387346, -295.1528744107228022, -342.9991450440437575 ) ) ;
#46331=CARTESIAN_POINT ( 'NONE',  ( -34.47897102602613728, -283.0170992835729749, -347.3078838800832386 ) ) ;
#46332=CARTESIAN_POINT ( 'NONE',  ( 38.19992841572207709, -283.4306793522565613, -267.0947722615724729 ) ) ;
#46333=CARTESIAN_POINT ( 'NONE',  ( 1.514672317913646982, -286.2233352209967165, -203.8933446736745339 ) ) ;
#46334=CARTESIAN_POINT ( 'NONE',  ( -108.7434333408032501, -288.8421187522321247, -247.9166387788759494 ) ) ;
#46336=CARTESIAN_POINT ( 'NONE',  ( 39.01674746887911738, -280.0268864339724360, -269.9534690223280222 ) ) ;
#46337=CARTESIAN_POINT ( 'NONE',  ( 38.25450449644097972, -286.3093869475776501, -257.3723007814103312 ) ) ;
#46339=CARTESIAN_POINT ( 'NONE',  ( -41.05935858943956873, -296.6998137170402288, -344.0801283360063394 ) ) ;
#46340=CARTESIAN_POINT ( 'NONE',  ( 35.93361755758476761, -277.2518259647716832, -292.0714397965968487 ) ) ;
#46341=CARTESIAN_POINT ( 'NONE',  ( 37.59338493961973171, -291.4645839810127654, -261.9354214932698142 ) ) ;
#46342=CARTESIAN_POINT ( 'NONE',  ( -38.34988255329290752, -279.7058919817886817, -197.3345298516230173 ) ) ;
#46343=CARTESIAN_POINT ( 'NONE',  ( 39.71161926582044543, -293.7181655676005789, -270.3078399084605508 ) ) ;
#46344=CARTESIAN_POINT ( 'NONE',  ( -107.6788896007015097, -282.9902236642016078, -242.6147070906043837 ) ) ;
#46346=CARTESIAN_POINT ( 'NONE',  ( -103.2067127041706698, -280.0757008774535848, -306.2331232843191628 ) ) ;
#46347=CARTESIAN_POINT ( 'NONE',  ( 17.24798155832381852, -293.3072305702777953, -319.1998442266411189 ) ) ;
#46348=CARTESIAN_POINT ( 'NONE',  ( -35.50665490957358372, -296.0749665335084728, -195.3617348925761235 ) ) ;
#46351=CARTESIAN_POINT ( 'NONE',  ( -57.58291125297170510, -281.7694366269533361, -198.5130827124814914 ) ) ;
#46352=CARTESIAN_POINT ( 'NONE',  ( 34.27805597506248603, -292.8694372884131099, -255.9181619983269513 ) ) ;
#46354=CARTESIAN_POINT ( 'NONE',  ( -53.28691492658257545, -295.3380690714490129, -200.3538533559491555 ) ) ;
#46355=CARTESIAN_POINT ( 'NONE',  ( -112.2835255618849999, -271.9619667686486650, -253.3940433356491440 ) ) ;
#46356=CARTESIAN_POINT ( 'NONE',  ( 35.91804928170274991, -289.1464020034975420, -292.4590311703821044 ) ) ;
#46357=CARTESIAN_POINT ( 'NONE',  ( 7.978283973949081620, -288.2458957510714299, -327.5895990516440861 ) ) ;
#46358=CARTESIAN_POINT ( 'NONE',  ( -88.02135643986768798, -280.8481165182821542, -216.7902964030737394 ) ) ;
#46359=CARTESIAN_POINT ( 'NONE',  ( -95.25809100411727570, -298.9541240556448543, -224.2778706503605690 ) ) ;
#46360=CARTESIAN_POINT ( 'NONE',  ( -59.84083681738145799, -278.5491162600953317, -200.4439503244655612 ) ) ;
#46362=CARTESIAN_POINT ( 'NONE',  ( 30.76934322675772293, -298.5497918239036039, -193.3859609996251265 ) ) ;
#46363=CARTESIAN_POINT ( 'NONE',  ( -11.78841591291329749, -294.3074546909768401, -200.3894926422692606 ) ) ;
#46364=CARTESIAN_POINT ( 'NONE',  ( 32.68947203243885724, -295.5403470442806224, -300.5290273544906654 ) ) ;
#46365=DIRECTION ( 'NONE',  ( 0.000000000000000000, 0.000000000000000000, -1.000000000000000000 ) ) ;
#46366=CARTESIAN_POINT ( 'NONE',  ( -110.4077740675563177, -291.1566586507199759, -273.9221826773558064 ) ) ;
#46368=CARTESIAN_POINT ( 'NONE',  ( 31.08082618801976338, -291.2665010447502141, -237.7020057178556840 ) ) ;
#46369=CARTESIAN_POINT ( 'NONE',  ( -99.91272315313989338, -296.7378393500935658, -232.6203390726961118 ) ) ;
#46372=CARTESIAN_POINT ( 'NONE',  ( -110.1147047664034773, -291.7792450655117023, -293.4856677743620708 ) ) ;
#46373=CARTESIAN_POINT ( 'NONE',  ( 40.65961533371913106, -296.2662352645559167, -288.1317622949166548 ) ) ;
#46374=CARTESIAN_POINT ( 'NONE',  ( 20.05185306690983182, -288.8871543897271863, -222.3202461236955685 ) ) ;
#46375=CARTESIAN_POINT ( 'NONE',  ( 16.79014183914382841, -272.8242979144181959, -218.6162415006879769 ) ) ;
#46376=CARTESIAN_POINT ( 'NONE',  ( 35.30383162187533941, -277.6832253726983026, -286.6654224065933931 ) ) ;
#46377=CARTESIAN_POINT ( 'NONE',  ( -44.41312411285835537, -290.0419883669500223, -196.2059303815636326 ) ) ;
#46378=CARTESIAN_POINT ( 'NONE',  ( -35.39194776999691783, -281.9367581745924554, -194.6084798188588536 ) ) ;
#46380=CARTESIAN_POINT ( 'NONE',  ( 3.440218207359738045, -281.8366552454165230, -331.0913462205418796 ) ) ;
#46381=CARTESIAN_POINT ( 'NONE',  ( -109.3208575026317391, -279.9693989404456147, -243.7408889201573174 ) ) ;
#46382=CARTESIAN_POINT ( 'NONE',  ( 37.15858708771732211, -280.5718154017666848, -288.2416088204408879 ) ) ;
#46383=CARTESIAN_POINT ( 'NONE',  ( -32.29525589772949701, -123.9253558744183010, -361.4536083058858935 ) ) ;
#46384=CARTESIAN_POINT ( 'NONE',  ( 13.79876679911920156, -275.6895075074633041, -213.0408770695811711 ) ) ;
#46387=CARTESIAN_POINT ( 'NONE',  ( 21.30545371755189876, -276.4096568132458174, -221.5428928950725833 ) ) ;
#46388=CARTESIAN_POINT ( 'NONE',  ( -110.4542110544635705, -298.8376638359844719, -287.0812184334320705 ) ) ;
#46392=CARTESIAN_POINT ( 'NONE',  ( -106.3187866098970176, -291.3025600349148476, -295.1882727475874049 ) ) ;
#46393=CARTESIAN_POINT ( 'NONE',  ( -88.78872062443217317, -291.5230351917008420, -326.2822954904153789 ) ) ;
#46394=CARTESIAN_POINT ( 'NONE',  ( -22.71213192228901079, -291.5929570822947312, -198.7380183432076990 ) ) ;
#46395=CARTESIAN_POINT ( 'NONE',  ( 1.496033748994984425, -286.0642948689919649, -203.9292471266118696 ) ) ;
#46397=CARTESIAN_POINT ( 'NONE',  ( -4.489142514825396724, -281.0116512783066014, -336.4455327542974601 ) ) ;
#46398=CARTESIAN_POINT ( 'NONE',  ( 36.91527576519431619, -289.3852435326124350, -268.2541570470018542 ) ) ;
#46399=CARTESIAN_POINT ( 'NONE',  ( 19.87824628872928656, -280.6831573958477861, -316.8200539764588370 ) ) ;
#46400=CARTESIAN_POINT ( 'NONE',  ( 35.04998085649585704, -282.7012311139661165, -257.6848408079382580 ) ) ;
#46401=CARTESIAN_POINT ( 'NONE',  ( 35.72747335436562111, -288.7902196797586498, -293.8922909122684359 ) ) ;
#46402=CARTESIAN_POINT ( 'NONE',  ( -107.6792578609853877, -279.3060782671766447, -250.5507162075596455 ) ) ;
#46403=CARTESIAN_POINT ( 'NONE',  ( -108.4356802373065420, -288.9832073504236973, -298.8857513700295385 ) ) ;
#46404=CARTESIAN_POINT ( 'NONE',  ( -95.70063300322010491, -286.0315078299092875, -220.2973688517673168 ) ) ;
#46405=CARTESIAN_POINT ( 'NONE',  ( 16.25182647336717068, -287.2810180583446140, -215.1591179323358460 ) ) ;
#46406=CARTESIAN_POINT ( 'NONE',  ( -105.2131509675829903, -284.3576376503070264, -297.3774390006513499 ) ) ;
#46409=CARTESIAN_POINT ( 'NONE',  ( 32.18141296128852957, -295.0225519098081577, -240.2472968312838759 ) ) ;
#46410=CARTESIAN_POINT ( 'NONE',  ( 38.95056213539505308, -292.1649048759869061, -264.6349508133022823 ) ) ;
#46411=CARTESIAN_POINT ( 'NONE',  ( -3.770250696512623456, -275.6565233490712217, -335.4484918104378721 ) ) ;
#46412=CARTESIAN_POINT ( 'NONE',  ( -41.94775898574346229, -294.4572157296943828, -347.1734380241659323 ) ) ;
#46413=CARTESIAN_POINT ( 'NONE',  ( -70.51565781845140179, -290.0863837760697947, -204.5568910248455836 ) ) ;
#46414=CARTESIAN_POINT ( 'NONE',  ( 8.843250423906901858, -292.6490410919157057, -328.2622899375991778 ) ) ;
#46415=CARTESIAN_POINT ( 'NONE',  ( -102.7704557630788145, -292.2078339740842239, -236.9888535220450478 ) ) ;
#46416=CARTESIAN_POINT ( 'NONE',  ( -3.505758968497529438, -293.5895482063708073, -205.3276253788006613 ) ) ;
#46418=CARTESIAN_POINT ( 'NONE',  ( -41.86140837607259613, -293.1086862304427996, -345.4429281183137164 ) ) ;
#46419=CARTESIAN_POINT ( 'NONE',  ( -44.00562195928616660, -299.9681931489901103, -195.6069440379329762 ) ) ;
#46420=CARTESIAN_POINT ( 'NONE',  ( -3.246179430729769333, -289.5318387246890666, -335.2316691412055434 ) ) ;
#46421=CARTESIAN_POINT ( 'NONE',  ( 24.72674802516062442, -278.1094940323442870, -313.1821945748203007 ) ) ;
#46422=CARTESIAN_POINT ( 'NONE',  ( -109.3686879415191555, -277.0142365354618619, -296.5955206070291297 ) ) ;
#46423=CARTESIAN_POINT ( 'NONE',  ( -87.96302347577335468, -272.7147809255042148, -212.4042825872313927 ) ) ;
#46424=CARTESIAN_POINT ( 'NONE',  ( 30.29103816560489193, -279.2191305179655956, -239.1388334326545362 ) ) ;
#46425=CARTESIAN_POINT ( 'NONE',  ( -77.41173809772131165, -275.9796151952839409, -335.2362731638159516 ) ) ;
#46426=CARTESIAN_POINT ( 'NONE',  ( -93.46979529053184876, -294.5670767082834232, -317.8240637294426847 ) ) ;
#46427=CARTESIAN_POINT ( 'NONE',  ( -68.51488237780591817, -275.6427384623713124, -202.1326231451482442 ) ) ;
#46428=CARTESIAN_POINT ( 'NONE',  ( -37.83384158578008538, -298.8486663569955795, -197.2012961926343451 ) ) ;
#46430=CARTESIAN_POINT ( 'NONE',  ( -86.33460885551939157, -287.7478770723640764, -327.6843844502901106 ) ) ;
#46431=CARTESIAN_POINT ( 'NONE',  ( 17.28696614175932567, -274.6928676796962918, -221.8640199470314940 ) ) ;
#46432=CARTESIAN_POINT ( 'NONE',  ( 18.64481637960401983, -288.2740710177165511, -323.2242428366080276 ) ) ;
#46433=CARTESIAN_POINT ( 'NONE',  ( -59.68497609087143019, -299.7441908903262515, -198.3402217715505174 ) ) ;
#46434=CARTESIAN_POINT ( 'NONE',  ( -112.0738212627230439, -294.5019180846687732, -274.2519398153865495 ) ) ;
#46435=CARTESIAN_POINT ( 'NONE',  ( 9.103058559264185945, -281.6296965013964382, -331.5742147060465186 ) ) ;
#46437=CARTESIAN_POINT ( 'NONE',  ( -8.292988324166739034, -280.6716752413627773, -339.5209101439962183 ) ) ;
#46439=CARTESIAN_POINT ( 'NONE',  ( -93.73512308261878445, -290.0101967664827498, -223.3637169999577736 ) ) ;
#46441=CARTESIAN_POINT ( 'NONE',  ( -108.5838958349923757, -282.4197322264703303, -291.2731555933654590 ) ) ;
#46444=CARTESIAN_POINT ( 'NONE',  ( -109.3073868082940123, -288.8244599757809965, -249.1982652254150423 ) ) ;
#46445=CARTESIAN_POINT ( 'NONE',  ( -0.2135237236779599368, -276.0756970226396447, -206.6894484954567588 ) ) ;
#46446=CARTESIAN_POINT ( 'NONE',  ( 11.13291786550620621, -283.8215966836567645, -329.4958146255698921 ) ) ;
#46447=CARTESIAN_POINT ( 'NONE',  ( -93.99037616140643081, -271.3220131083025990, -220.3587010078310300 ) ) ;
#46448=CARTESIAN_POINT ( 'NONE',  ( -37.54052282974512877, -283.0547449011847903, -343.3732765808597946 ) ) ;
#46449=CARTESIAN_POINT ( 'NONE',  ( 35.42156444521238967, -276.8324453484163996, -259.2818236959449223 ) ) ;
#46450=CARTESIAN_POINT ( 'NONE',  ( 35.80413762342946882, -276.3350792790271271, -268.8484560705453532 ) ) ;
#46451=EDGE_CURVE ( 'NONE', #17445, #36646, #79889, .T. ) ;
#46452=CARTESIAN_POINT ( 'NONE',  ( -64.50349158034769914, -285.4068306240286574, -340.2837322389356700 ) ) ;
#46454=CARTESIAN_POINT ( 'NONE',  ( 204.7719119196574411, 293.0780843197346144, -54.00000000000338929 ) ) ;
#46455=CARTESIAN_POINT ( 'NONE',  ( 1.767606473776451192, -294.3774121009295754, -336.6895594057350536 ) ) ;
#46456=CARTESIAN_POINT ( 'NONE',  ( -41.43784094566748877, -287.9802400865987693, -195.8160067305347525 ) ) ;
#46458=CARTESIAN_POINT ( 'NONE',  ( -19.05039376806006857, -283.7666405000204009, -190.3683826091709363 ) ) ;
#46459=CARTESIAN_POINT ( 'NONE',  ( -67.65433532881492340, -276.6370755009165237, -340.9677959104295155 ) ) ;
#46460=CARTESIAN_POINT ( 'NONE',  ( -64.08870748035188569, -290.1090029215429240, -198.9540250563174766 ) ) ;
#46461=CARTESIAN_POINT ( 'NONE',  ( -54.94050206904025657, -287.3420280703763297, -198.7472279257920604 ) ) ;
#46462=CARTESIAN_POINT ( 'NONE',  ( -76.87844364834829491, -279.3492813123046403, -332.9899053948845449 ) ) ;
#46463=CARTESIAN_POINT ( 'NONE',  ( -70.82453441366230606, -287.0443459470996004, -201.6770142629244731 ) ) ;
#46464=CARTESIAN_POINT ( 'NONE',  ( 6.788913995194937989, -284.4519230579898021, -331.0034261761716721 ) ) ;
#46465=CARTESIAN_POINT ( 'NONE',  ( 39.63080533149643969, -275.6930996702062657, -268.3035933143937655 ) ) ;
#46466=CARTESIAN_POINT ( 'NONE',  ( -34.29321983966458021, -276.8481353538730900, -347.3007486838610589 ) ) ;
#46467=CARTESIAN_POINT ( 'NONE',  ( -103.8292990821091593, -298.9192201444915895, -236.7692148447806915 ) ) ;
#46470=CARTESIAN_POINT ( 'NONE',  ( -57.04528014716949258, -295.9403570344323953, -197.1488575668585952 ) ) ;
#46472=CARTESIAN_POINT ( 'NONE',  ( -110.3418825866378654, -278.0203441884185054, -273.3547449623461603 ) ) ;
#46473=CARTESIAN_POINT ( 'NONE',  ( 4.632690563354548097, -275.8098827084253912, -206.2188701014767105 ) ) ;
#46474=CARTESIAN_POINT ( 'NONE',  ( 37.75698957542275025, -280.4105768394371125, -254.3919926805629075 ) ) ;
#46475=CARTESIAN_POINT ( 'NONE',  ( -6.616002688921249764, -288.2213426497713726, -203.0129209775155630 ) ) ;
#46476=CARTESIAN_POINT ( 'NONE',  ( -113.6721291979071111, -298.0456576170525409, -272.4701219602595756 ) ) ;
#46477=CARTESIAN_POINT ( 'NONE',  ( -64.11296887098848174, -296.5988460454856863, -342.1337303653332924 ) ) ;
#46479=CARTESIAN_POINT ( 'NONE',  ( 24.07845450243603125, -294.9707634450836053, -227.5881933692811856 ) ) ;
#46480=CARTESIAN_POINT ( 'NONE',  ( -41.11887304149887967, -278.0043305840779908, -195.6231664915185604 ) ) ;
#46481=CARTESIAN_POINT ( 'NONE',  ( -2.496257393005111069, -282.4369078404466791, -204.5658955737301881 ) ) ;
#46482=CARTESIAN_POINT ( 'NONE',  ( -108.8357003007970292, -294.9009456538357767, -249.6265541226763105 ) ) ;
#46483=CARTESIAN_POINT ( 'NONE',  ( -102.2260972412861690, -285.6245452182780582, -310.3167862361407288 ) ) ;
#46484=CARTESIAN_POINT ( 'NONE',  ( 19.76461015206173144, -285.8251067063666255, -224.3728071224861367 ) ) ;
#46485=CARTESIAN_POINT ( 'NONE',  ( 1.329898937396618352, -279.9027848580465729, -203.8338049045802052 ) ) ;
#46486=CARTESIAN_POINT ( 'NONE',  ( -61.77620294925019806, -183.7782069458722845, -361.8444782285974384 ) ) ;
#46488=CARTESIAN_POINT ( 'NONE',  ( -14.55537852441836044, -286.0223818072741437, -200.9332241126281815 ) ) ;
#46490=CARTESIAN_POINT ( 'NONE',  ( -34.47669755257052060, -284.0965961714980494, -346.9984735655148143 ) ) ;
#46491=CARTESIAN_POINT ( 'NONE',  ( 34.72872807739076961, -276.0443542757327009, -282.4115702967845891 ) ) ;
#46492=CARTESIAN_POINT ( 'NONE',  ( 26.03751117941197180, -285.7766374851220803, -227.3134500792251060 ) ) ;
#46493=CARTESIAN_POINT ( 'NONE',  ( -81.74019806730593984, -290.3833181852807570, -207.8289991177871059 ) ) ;
#46494=CARTESIAN_POINT ( 'NONE',  ( 35.94749142148326371, -282.2056294564739005, -247.5244234982417026 ) ) ;
#46496=CARTESIAN_POINT ( 'NONE',  ( -14.45433086940533407, -281.8635802459497768, -197.5123465187869272 ) ) ;
#46497=CARTESIAN_POINT ( 'NONE',  ( 34.30318578081588754, -281.5267522505560009, -242.0597524498827795 ) ) ;
#46498=CARTESIAN_POINT ( 'NONE',  ( -105.5937364680635966, -281.8380690714489560, -285.9065529553535612 ) ) ;
#46499=CARTESIAN_POINT ( 'NONE',  ( -47.47154897853537392, -155.3119904466320804, -365.2842717752373574 ) ) ;
#46501=CARTESIAN_POINT ( 'NONE',  ( 35.02136117726902853, -277.7979341047210369, -289.4298302571585850 ) ) ;
#46502=CARTESIAN_POINT ( 'NONE',  ( 188.7542133104363415, 271.4570962582653806, -139.3427320832213638 ) ) ;
#46503=CARTESIAN_POINT ( 'NONE',  ( 37.20737500415631160, -279.6210096644622354, -274.1402973787165251 ) ) ;
#46504=CARTESIAN_POINT ( 'NONE',  ( -81.99984057473265864, -296.7738103376374283, -212.4217306007535342 ) ) ;
#46505=CARTESIAN_POINT ( 'NONE',  ( -79.55540984551448958, -291.0063263815785035, -205.9738042515697600 ) ) ;
#46508=CARTESIAN_POINT ( 'NONE',  ( -80.27880545019738179, -296.0581093270862425, -207.0914089845376509 ) ) ;
#46509=CARTESIAN_POINT ( 'NONE',  ( 20.15111980897052035, -285.3047340312012352, -224.0699744219512866 ) ) ;
#46510=CARTESIAN_POINT ( 'NONE',  ( 34.31511994998453474, -295.6650723877946234, -289.8044982718808456 ) ) ;
#46511=EDGE_CURVE ( 'NONE', #21957, #78913, #27248, .T. ) ;
#46512=CARTESIAN_POINT ( 'NONE',  ( 9.330855014310634132, -288.0245267162670189, -213.5903854431656157 ) ) ;
#46514=CARTESIAN_POINT ( 'NONE',  ( 37.23428988671186346, -294.7223839500972531, -288.6162091161399417 ) ) ;
#46515=CARTESIAN_POINT ( 'NONE',  ( -106.5926498419017463, -285.3554628579443033, -246.9154461683848467 ) ) ;
#46516=CARTESIAN_POINT ( 'NONE',  ( -103.4990952029686753, -295.8533586527062198, -231.6404577125566391 ) ) ;
#46517=CARTESIAN_POINT ( 'NONE',  ( -8.581166271665804146, -293.2219674376185026, -199.1081144466369039 ) ) ;
#46518=CARTESIAN_POINT ( 'NONE',  ( -34.96859767793201001, -292.5735202635398764, -193.4461234652441135 ) ) ;
#46519=CARTESIAN_POINT ( 'NONE',  ( -13.28587243346614066, -288.8974840554821526, -339.2836626136479481 ) ) ;
#46520=ORIENTED_EDGE ( 'NONE', *, *, #74502, .T. ) ;
#46522=CARTESIAN_POINT ( 'NONE',  ( -9.696521646170193520, -300.2551450493016318, -194.5876580512280327 ) ) ;
#46523=CARTESIAN_POINT ( 'NONE',  ( -106.4782272792930655, -271.7721689242761158, -237.3740094259029547 ) ) ;
#46524=CARTESIAN_POINT ( 'NONE',  ( -32.14091564159048175, -282.0436832783194632, -343.4115135259049225 ) ) ;
#46526=CARTESIAN_POINT ( 'NONE',  ( -34.29980923948419047, -276.5225208320015327, -347.2394231356013279 ) ) ;
#46527=CARTESIAN_POINT ( 'NONE',  ( -91.69812366915154200, -271.6608971428851191, -220.4242877252961819 ) ) ;
#46528=CARTESIAN_POINT ( 'NONE',  ( -107.6216710325976607, -280.7268517594920354, -246.2951353709926821 ) ) ;
#46529=CARTESIAN_POINT ( 'NONE',  ( 32.41443528281216402, -274.0262437218823379, -295.9061690981015431 ) ) ;
#46530=CARTESIAN_POINT ( 'NONE',  ( -69.44499153016444382, -298.8249977409690814, -204.3572606151357149 ) ) ;
#46531=CARTESIAN_POINT ( 'NONE',  ( -39.18984574589416070, -299.1081261503075552, -197.0628434366063004 ) ) ;
#46532=CARTESIAN_POINT ( 'NONE',  ( -112.1077475633819205, -298.3390650588717676, -255.5807153435105761 ) ) ;
#46533=CARTESIAN_POINT ( 'NONE',  ( -29.97406864047778541, -272.1650794284279300, -195.3669528197211775 ) ) ;
#46534=CARTESIAN_POINT ( 'NONE',  ( 1.631185191535880374, -295.1677828401715828, -332.2677131690297756 ) ) ;
#46535=CARTESIAN_POINT ( 'NONE',  ( -60.42672580765761126, -290.3216947233413521, -200.4330781412546685 ) ) ;
#46537=CARTESIAN_POINT ( 'NONE',  ( 11.74160832447875613, -275.2047662835769870, -211.0436376925225090 ) ) ;
#46538=CARTESIAN_POINT ( 'NONE',  ( -110.3417001280813707, -272.7188053858000671, -270.3632352445363267 ) ) ;
#46539=CARTESIAN_POINT ( 'NONE',  ( 30.63128665182165022, -280.6925371517787084, -305.4748096095851793 ) ) ;
#46541=CARTESIAN_POINT ( 'NONE',  ( -87.04602165081868748, -282.9625272965397471, -324.1154638808611708 ) ) ;
#46542=CARTESIAN_POINT ( 'NONE',  ( -35.95908338051339825, -281.0347259743611517, -345.5278769504558909 ) ) ;
#46543=CARTESIAN_POINT ( 'NONE',  ( -9.784421121998015280, -275.2597489329264135, -338.6094696337240180 ) ) ;
#46544=CARTESIAN_POINT ( 'NONE',  ( 24.52240164543244560, -284.1277778642296425, -312.8511540795840347 ) ) ;
#46549=CARTESIAN_POINT ( 'NONE',  ( -64.59472941738422946, -272.1021126672830519, -199.1873117509834685 ) ) ;
#46550=CARTESIAN_POINT ( 'NONE',  ( -112.2497287703827169, -280.4648215103738380, -277.1904708549156453 ) ) ;
#46552=CARTESIAN_POINT ( 'NONE',  ( -98.60628917152341444, -285.8736722264678178, -314.6748056152290474 ) ) ;
#46555=CARTESIAN_POINT ( 'NONE',  ( -90.35999277721030865, -287.8018218744213641, -323.4812491160253103 ) ) ;
#46557=CARTESIAN_POINT ( 'NONE',  ( -88.79107481039878280, -294.5888948618323866, -322.7784501479519008 ) ) ;
#46558=CARTESIAN_POINT ( 'NONE',  ( -87.58248017972501032, -287.9015490681890697, -325.0818535784466121 ) ) ;
#46559=CARTESIAN_POINT ( 'NONE',  ( -99.29329069375972949, -236.7418906163237580, -339.9611904871904358 ) ) ;
#46560=CARTESIAN_POINT ( 'NONE',  ( -112.0948556754403427, -294.4660598399690343, -277.0534350092479485 ) ) ;
#46561=CARTESIAN_POINT ( 'NONE',  ( 38.39989222181901596, -286.1543634083397478, -280.0544876338055360 ) ) ;
#46562=CARTESIAN_POINT ( 'NONE',  ( 36.22828717972275570, -283.2363178523491456, -276.8008891564444411 ) ) ;
#46563=CARTESIAN_POINT ( 'NONE',  ( -3.366303541904547725, -280.8496913973339133, -338.3435576598768080 ) ) ;
#46564=CARTESIAN_POINT ( 'NONE',  ( 12.15580102355880854, -288.3406755816164377, -324.0860959863687185 ) ) ;
#46565=CARTESIAN_POINT ( 'NONE',  ( 30.88757684273510407, -283.3436705467093475, -297.9317668663750851 ) ) ;
#46566=CARTESIAN_POINT ( 'NONE',  ( 28.30045861956977404, -282.7931657773804091, -302.7826016632959067 ) ) ;
#46567=CARTESIAN_POINT ( 'NONE',  ( 27.27488020807414415, -289.0142107210244831, -231.4906465224462124 ) ) ;
#46569=CARTESIAN_POINT ( 'NONE',  ( -30.48671247894817427, -298.3024367115428959, -193.3609299358889473 ) ) ;
#46571=CARTESIAN_POINT ( 'NONE',  ( -99.56705243431393626, -273.1551104488721649, -224.9184825532749983 ) ) ;
#46572=CARTESIAN_POINT ( 'NONE',  ( 7.647966158127728953, -294.6495862211684766, -210.7979017570939959 ) ) ;
#46574=CARTESIAN_POINT ( 'NONE',  ( -106.6662871844225293, -281.4805209788417528, -237.0123917617630980 ) ) ;
#46576=CARTESIAN_POINT ( 'NONE',  ( -8.609558829170946836, -274.6768893165237273, -339.8336268800298967 ) ) ;
#46578=CARTESIAN_POINT ( 'NONE',  ( -113.5378019297075554, -294.9617684197314702, -269.5900903333194378 ) ) ;
#46579=CARTESIAN_POINT ( 'NONE',  ( -16.60381347833856225, -273.6757199202681363, -200.2095983897104645 ) ) ;
#46580=CARTESIAN_POINT ( 'NONE',  ( -75.35367709335112352, -293.0559306613838544, -207.1683618300355079 ) ) ;
#46581=CARTESIAN_POINT ( 'NONE',  ( -93.62834761314395848, -292.1561772618987902, -223.4883427569804724 ) ) ;
#46582=CARTESIAN_POINT ( 'NONE',  ( 19.28391228345673625, -283.9802102709580254, -318.0412025849864790 ) ) ;
#46583=CARTESIAN_POINT ( 'NONE',  ( -113.2261450943129262, -291.8590950070779400, -279.7500239434645550 ) ) ;
#46584=CARTESIAN_POINT ( 'NONE',  ( -42.04051370237161933, -293.3092564129298694, -193.9986964379793051 ) ) ;
#46585=CARTESIAN_POINT ( 'NONE',  ( -26.20950126106492561, -294.7397945242577180, -342.5073178330993073 ) ) ;
#46586=CARTESIAN_POINT ( 'NONE',  ( 21.95394524892376609, -290.1820178921375941, -316.3060666026779018 ) ) ;
#46587=CARTESIAN_POINT ( 'NONE',  ( 28.30611449797990886, -282.2457496656749640, -310.7034942541572491 ) ) ;
#46588=CARTESIAN_POINT ( 'NONE',  ( -94.50836201296606021, -293.9518631375467521, -319.7704993705849574 ) ) ;
#46589=CARTESIAN_POINT ( 'NONE',  ( -31.63840623613665315, -282.8153818476476431, -347.1628775364534363 ) ) ;
#46590=CARTESIAN_POINT ( 'NONE',  ( 1.753912904981421050, -278.5068207043474899, -334.0094404234041576 ) ) ;
#46591=CARTESIAN_POINT ( 'NONE',  ( -108.5835401312018291, -276.3590019111426273, -296.3004918719157104 ) ) ;
#46593=CARTESIAN_POINT ( 'NONE',  ( 15.86637979916431362, -281.7807001949903452, -320.5029402491841779 ) ) ;
#46594=CARTESIAN_POINT ( 'NONE',  ( -41.00483948908105702, -281.2121194942228044, -193.8326971583397835 ) ) ;
#46595=CARTESIAN_POINT ( 'NONE',  ( 9.676121556389981393, -285.7402886695355733, -209.6804401985278616 ) ) ;
#46596=CARTESIAN_POINT ( 'NONE',  ( -66.99030088293672236, -293.4182639793105523, -202.5456736602772310 ) ) ;
#46597=CARTESIAN_POINT ( 'NONE',  ( 37.70066684158338433, -276.9841144675755231, -257.0547561907097815 ) ) ;
#46598=CARTESIAN_POINT ( 'NONE',  ( 38.23780358342659724, -276.7167789953472834, -258.4008937734320739 ) ) ;
#46599=CARTESIAN_POINT ( 'NONE',  ( -108.4867444995050931, -278.1690329238269896, -286.7683621450599389 ) ) ;
#46600=CARTESIAN_POINT ( 'NONE',  ( -111.2142068344568173, -274.6747812398086808, -259.2972781682528876 ) ) ;
#46601=CARTESIAN_POINT ( 'NONE',  ( 37.43845261011856707, -293.4480569937410905, -288.6829804417172340 ) ) ;
#46602=CARTESIAN_POINT ( 'NONE',  ( -97.51519561589029195, -291.5213448295623380, -317.1114212866702928 ) ) ;
#46603=CARTESIAN_POINT ( 'NONE',  ( -14.73808618523979774, -291.2723928470009582, -200.6237341069408728 ) ) ;
#46605=CARTESIAN_POINT ( 'NONE',  ( -66.56864206318293498, -291.3251799890189773, -203.4442041867044111 ) ) ;
#46607=CARTESIAN_POINT ( 'NONE',  ( -36.07809076639345847, -290.1163566599614114, -347.0546541457024432 ) ) ;
#46608=CARTESIAN_POINT ( 'NONE',  ( -39.71283842052467605, -280.6730390831329487, -197.2851126979471132 ) ) ;
#46609=CARTESIAN_POINT ( 'NONE',  ( -104.9744953429309078, -295.9429009894870433, -234.0919320306861948 ) ) ;
#46610=CARTESIAN_POINT ( 'NONE',  ( 2.680869986122784265, -287.2255899567784354, -204.6990538363054952 ) ) ;
#46611=CARTESIAN_POINT ( 'NONE',  ( 33.83825483885439667, -287.5112753461085617, -240.9104792703699616 ) ) ;
#46613=CARTESIAN_POINT ( 'NONE',  ( -95.93617238407178149, -284.2743898774062359, -313.9360569714524445 ) ) ;
#46614=CARTESIAN_POINT ( 'NONE',  ( -56.47922461787481296, -169.2600705521303155, -364.3876518943077372 ) ) ;
#46615=CARTESIAN_POINT ( 'NONE',  ( 43.60372932191738471, 12.79097968492800419, -330.4845513384636888 ) ) ;
#46616=CARTESIAN_POINT ( 'NONE',  ( 160.0134857714809868, 218.2058721980534131, -202.3628264432244350 ) ) ;
#46617=CARTESIAN_POINT ( 'NONE',  ( -89.20749389083766800, -277.0018624060468255, -322.0328857616854066 ) ) ;
#46618=CARTESIAN_POINT ( 'NONE',  ( 35.89657587248282056, -274.4169574217511354, -266.1347974990356420 ) ) ;
#46619=CARTESIAN_POINT ( 'NONE',  ( -114.1596139752474812, -272.2906471836773790, -264.6235902141106067 ) ) ;
#46620=CARTESIAN_POINT ( 'NONE',  ( 104.1431745715192108, 114.1911308902789131, -280.0153630978813908 ) ) ;
#46622=CARTESIAN_POINT ( 'NONE',  ( -110.2022031407864944, -276.9397264110240826, -293.8694482995268231 ) ) ;
#46623=CARTESIAN_POINT ( 'NONE',  ( -105.3191693759786176, -274.7018240896084649, -240.9559402438141262 ) ) ;
#46625=CARTESIAN_POINT ( 'NONE',  ( -106.0883560879463232, -290.7153304748176197, -295.0974422026754382 ) ) ;
#46626=CARTESIAN_POINT ( 'NONE',  ( -23.40650237791145116, -299.0252869540051961, -193.5207482409714714 ) ) ;
#46627=CARTESIAN_POINT ( 'NONE',  ( -75.75462430054365370, -298.0464484496349087, -203.6368322189051412 ) ) ;
#46628=CARTESIAN_POINT ( 'NONE',  ( 17.08198505742569751, -294.4149836624684440, -319.0324314909709074 ) ) ;
#46630=CARTESIAN_POINT ( 'NONE',  ( -5.861986287342172197, -278.5616776875972391, -339.0513051859056191 ) ) ;
#46631=CARTESIAN_POINT ( 'NONE',  ( -38.73772207297331960, -282.5768779335834324, -347.2869135665104068 ) ) ;
#46632=CARTESIAN_POINT ( 'NONE',  ( -109.0643579511549603, -279.4325707987173359, -285.5297180951608311 ) ) ;
#46633=CARTESIAN_POINT ( 'NONE',  ( 9.913641704785165487, -278.1719366065626673, -329.9338413607540588 ) ) ;
#46634=CARTESIAN_POINT ( 'NONE',  ( -68.27882090709577767, -296.2123935670972514, -203.5770705003258172 ) ) ;
#46636=CARTESIAN_POINT ( 'NONE',  ( -96.88446650811557959, -278.1288498162246015, -312.6162137463947488 ) ) ;
#46637=CARTESIAN_POINT ( 'NONE',  ( -36.95084140150425611, -274.8597892339802229, -193.5105632280675536 ) ) ;
#46638=CARTESIAN_POINT ( 'NONE',  ( -40.33633225810174849, -287.7738592789223162, -346.8223364624061560 ) ) ;
#46639=CARTESIAN_POINT ( 'NONE',  ( -34.21280475890486628, -276.0916655243986497, -195.4264086363318995 ) ) ;
#46640=CARTESIAN_POINT ( 'NONE',  ( 39.04232645707350713, -274.1014035657841532, -268.3395408849036698 ) ) ;
#46642=CARTESIAN_POINT ( 'NONE',  ( -71.25667532229101653, -288.7090670983927794, -335.2010096735273237 ) ) ;
#46643=CARTESIAN_POINT ( 'NONE',  ( -114.1071690859248378, -283.8338513835529398, -275.7024244056433986 ) ) ;
#46644=CARTESIAN_POINT ( 'NONE',  ( 34.92505048358838593, -279.9999797905764467, -286.3451967039497958 ) ) ;
#46645=CARTESIAN_POINT ( 'NONE',  ( 31.90291973362528211, -280.4577649308583318, -295.4226713768119907 ) ) ;
#46646=CARTESIAN_POINT ( 'NONE',  ( -106.9020194466564675, -282.9790879706035867, -243.8530782145600710 ) ) ;
#46647=CARTESIAN_POINT ( 'NONE',  ( -104.7344854773557188, -292.1171017490884765, -303.3901034200227400 ) ) ;
#46648=CARTESIAN_POINT ( 'NONE',  ( -106.6340168383098899, -279.4352169025285093, -294.7165126826161554 ) ) ;
#46650=CARTESIAN_POINT ( 'NONE',  ( -63.65507890920710565, -281.7894108878634825, -341.8736799001981126 ) ) ;
#46651=CARTESIAN_POINT ( 'NONE',  ( 36.86904808483186713, -295.4085114551244828, -259.1614731028344636 ) ) ;
#46652=CARTESIAN_POINT ( 'NONE',  ( -56.28211438996942206, -278.0513834950457976, -196.7185677521244145 ) ) ;
#46653=CARTESIAN_POINT ( 'NONE',  ( -46.99507195992543274, -285.1746618724193922, -344.9053386650672337 ) ) ;
#46655=CARTESIAN_POINT ( 'NONE',  ( -103.8761969678313477, -292.0004431222741914, -306.1727770573348835 ) ) ;
#46656=CARTESIAN_POINT ( 'NONE',  ( 25.41913416240550916, -286.1612057914416596, -226.0074409139718057 ) ) ;
#46657=CARTESIAN_POINT ( 'NONE',  ( -38.89420052928657157, -290.4322239426742840, -196.5774466202844053 ) ) ;
#46659=CARTESIAN_POINT ( 'NONE',  ( 18.67349055953226866, -274.9089592096100318, -317.9378128175799247 ) ) ;
#46660=CARTESIAN_POINT ( 'NONE',  ( -34.27346081750354045, -293.1527472614341150, -344.5328874755946345 ) ) ;
#46663=CARTESIAN_POINT ( 'NONE',  ( 22.57580596936763229, -291.3941324423157084, -223.0898318017452198 ) ) ;
#46664=CARTESIAN_POINT ( 'NONE',  ( -77.50130454998196683, -287.1039550906161253, -208.3840265463012145 ) ) ;
#46665=CARTESIAN_POINT ( 'NONE',  ( -40.32175890250741190, -287.3289639892508376, -346.3022385609456251 ) ) ;
#46666=CARTESIAN_POINT ( 'NONE',  ( 9.390807003501517869, -288.1346072790750554, -213.5152941022397783 ) ) ;
#46668=CARTESIAN_POINT ( 'NONE',  ( 14.20438381706701314, -289.1077625939840345, -322.2803144007839364 ) ) ;
#46669=CARTESIAN_POINT ( 'NONE',  ( 35.48630691864657649, -295.2838994834227719, -250.9597017114630830 ) ) ;
#46672=CARTESIAN_POINT ( 'NONE',  ( 4.947616718786922441, -287.8146017465406885, -206.4260243713895306 ) ) ;
#46673=CARTESIAN_POINT ( 'NONE',  ( -96.81099048729556955, -275.9970493877451077, -316.9735380710748132 ) ) ;
#46674=CARTESIAN_POINT ( 'NONE',  ( -41.37909123622963392, -277.4349307691293234, -347.2472297835606128 ) ) ;
#46675=CARTESIAN_POINT ( 'NONE',  ( -14.28220519702349023, -290.4285825203360787, -198.3508233262575402 ) ) ;
#46676=CARTESIAN_POINT ( 'NONE',  ( -75.00793408253187522, -279.5646736540456914, -203.2026872408534359 ) ) ;
#46677=CARTESIAN_POINT ( 'NONE',  ( -94.89760861249123991, -299.1911398577760792, -222.8105603503004204 ) ) ;
#46679=CARTESIAN_POINT ( 'NONE',  ( -109.2658526243514672, -282.8278768411228725, -248.9228722796012505 ) ) ;
#46681=CARTESIAN_POINT ( 'NONE',  ( -107.6063063982399086, -277.0066196533318248, -246.2503205628196383 ) ) ;
#46682=CARTESIAN_POINT ( 'NONE',  ( 28.96584730303280963, -279.0860963705572999, -235.2030773423830396 ) ) ;
#46684=CARTESIAN_POINT ( 'NONE',  ( 20.28382865853616579, -274.7143387070482277, -320.4009455897826228 ) ) ;
#46685=CARTESIAN_POINT ( 'NONE',  ( -111.0683352647907753, -298.0935084864881333, -268.7367482327626931 ) ) ;
#46686=CARTESIAN_POINT ( 'NONE',  ( -8.169255774653347402, -281.5994052134367394, -341.3431679827423864 ) ) ;
#46687=CARTESIAN_POINT ( 'NONE',  ( -110.2858228500285662, -297.5864049509891629, -263.2888161205055439 ) ) ;
#46688=CARTESIAN_POINT ( 'NONE',  ( -112.6566200674386806, -298.0366440087377669, -256.9089394205408325 ) ) ;
#46689=CARTESIAN_POINT ( 'NONE',  ( -46.17713153867786247, -273.6036958065105296, -197.8764807238676156 ) ) ;
#46690=CARTESIAN_POINT ( 'NONE',  ( 22.57668471328187465, -294.9357139609228398, -225.2524956371835003 ) ) ;
#46691=CARTESIAN_POINT ( 'NONE',  ( 39.70250112861683789, -287.7336901139755128, -271.5491702985265761 ) ) ;
#46692=CARTESIAN_POINT ( 'NONE',  ( -112.6071379406231188, -276.7241942098969503, -263.1270051354865132 ) ) ;
#46693=CARTESIAN_POINT ( 'NONE',  ( -95.65952686948801897, -291.0646077996743202, -220.0614357714437972 ) ) ;
#46694=CARTESIAN_POINT ( 'NONE',  ( 16.15450826230483727, -285.8935200104600085, -220.3269695680680513 ) ) ;
#46695=CARTESIAN_POINT ( 'NONE',  ( -55.67460081037683750, -289.8161491580938218, -197.5827413428565649 ) ) ;
#46697=CARTESIAN_POINT ( 'NONE',  ( 24.80950920047307307, -22.49099280560490399, -345.4124233396505019 ) ) ;
#46698=CARTESIAN_POINT ( 'NONE',  ( -58.71311437851345971, -288.8436439243002951, -340.2799190209283324 ) ) ;
#46700=CARTESIAN_POINT ( 'NONE',  ( -89.73443779016372446, -286.2760793483358839, -214.1833619613309168 ) ) ;
#46701=CARTESIAN_POINT ( 'NONE',  ( 34.24775278838919945, -292.2571528448036702, -242.5054902150876615 ) ) ;
#46702=CARTESIAN_POINT ( 'NONE',  ( 16.64182079220857347, -282.4041863108669759, -216.5077882062450385 ) ) ;
#46703=CARTESIAN_POINT ( 'NONE',  ( -1.382128565355458694, -281.8340925258497691, -202.8318096285994159 ) ) ;
#46704=CARTESIAN_POINT ( 'NONE',  ( -32.14781935606998786, -282.8181302018990664, -343.1761137391787315 ) ) ;
#46705=CARTESIAN_POINT ( 'NONE',  ( -111.2153881658450416, -296.2792015064840712, -292.1257786404678995 ) ) ;
#46706=CARTESIAN_POINT ( 'NONE',  ( -68.50683993270271799, -274.9490711843843087, -203.7892500557035760 ) ) ;
#46707=CARTESIAN_POINT ( 'NONE',  ( 19.75054632130364496, -290.9041815193578486, -222.2745065287639079 ) ) ;
#46708=CARTESIAN_POINT ( 'NONE',  ( -36.46502778714970816, -296.9837068221518166, -197.0521690192059054 ) ) ;
#46711=CARTESIAN_POINT ( 'NONE',  ( -93.63231911263713414, -285.7914550963929514, -319.0906752722166857 ) ) ;
#46712=CARTESIAN_POINT ( 'NONE',  ( 4.071992744360424687, -295.5882287311251844, -334.9712940604021014 ) ) ;
#46713=CARTESIAN_POINT ( 'NONE',  ( -94.20656074971103067, -285.8525113270188740, -224.4034884059300623 ) ) ;
#46715=CARTESIAN_POINT ( 'NONE',  ( 23.32470423266149240, -275.2411354751882300, -317.4186696975211817 ) ) ;
#46716=CARTESIAN_POINT ( 'NONE',  ( 30.80474116737842749, -293.7419871243301372, -234.6182148998019557 ) ) ;
#46717=CARTESIAN_POINT ( 'NONE',  ( 0.9187094753207517561, -284.6964468662071113, -204.9514780428838208 ) ) ;
#46718=CARTESIAN_POINT ( 'NONE',  ( -4.616987851408536514, -292.8048746146095596, -200.6844540407172133 ) ) ;
#46719=CARTESIAN_POINT ( 'NONE',  ( -108.9586352519391852, -290.6966462182868440, -284.6764448294320005 ) ) ;
#46722=CARTESIAN_POINT ( 'NONE',  ( -101.8397201137918273, -254.3509017731851429, -324.1331500758875563 ) ) ;
#46723=CARTESIAN_POINT ( 'NONE',  ( -106.3701399115108615, -285.6518744641234093, -302.8846825465999473 ) ) ;
#46724=CARTESIAN_POINT ( 'NONE',  ( 31.09738932201053885, -296.4086741954486115, -195.3901485728259502 ) ) ;
#46726=CARTESIAN_POINT ( 'NONE',  ( -21.33405164084337713, -281.7624509208380914, -341.9534166131051052 ) ) ;
#46727=CARTESIAN_POINT ( 'NONE',  ( -111.3157526888499831, -278.4859703168679061, -249.0636101637744559 ) ) ;
#46728=CARTESIAN_POINT ( 'NONE',  ( -84.61512365627537235, -281.3998237904342545, -212.2832385099890189 ) ) ;
#46729=CARTESIAN_POINT ( 'NONE',  ( -101.3712253486714729, -256.2545489327123391, -325.4733069935736012 ) ) ;
#46730=CARTESIAN_POINT ( 'NONE',  ( -63.72572039728786564, -281.9642387780498325, -342.0722730902862168 ) ) ;
#46731=CARTESIAN_POINT ( 'NONE',  ( 5.693782458913366540, -284.6580936043405359, -209.3077381165867905 ) ) ;
#46732=CARTESIAN_POINT ( 'NONE',  ( -46.03646689318789242, -299.7034568587974377, -194.8735359340652735 ) ) ;
#46733=CARTESIAN_POINT ( 'NONE',  ( -102.8205296441016259, -296.6041395492026140, -302.8870183449707838 ) ) ;
#46735=CARTESIAN_POINT ( 'NONE',  ( 30.31625490522999655, -291.8527042035598242, -241.5316400211297605 ) ) ;
#46736=CARTESIAN_POINT ( 'NONE',  ( -6.607810289531760972, -277.3105137605671189, -340.8646517337873547 ) ) ;
#46737=CARTESIAN_POINT ( 'NONE',  ( 27.86128662085983976, -275.1066291771242618, -237.5347487191553739 ) ) ;
#46738=CARTESIAN_POINT ( 'NONE',  ( 38.61990525563883381, -274.3399952410734386, -259.8099560949489728 ) ) ;
#46740=CARTESIAN_POINT ( 'NONE',  ( -95.56402688411247937, -271.2033622209871169, -223.0637146685942866 ) ) ;
#46742=CARTESIAN_POINT ( 'NONE',  ( -2.222015681115426133, -296.0217567322440573, -338.2228454791646186 ) ) ;
#46746=CARTESIAN_POINT ( 'NONE',  ( -107.2766376429477901, -285.3416583648190112, -292.3458988216260650 ) ) ;
#46747=CARTESIAN_POINT ( 'NONE',  ( 23.76334358981527473, -282.7039803391659234, -225.1931243597964283 ) ) ;
#46748=CARTESIAN_POINT ( 'NONE',  ( -94.36973702319804147, -283.2551381691380357, -316.1160935256242510 ) ) ;
#46749=CARTESIAN_POINT ( 'NONE',  ( -8.443999797408698882, -275.0673268475259761, -338.2818266226420292 ) ) ;
#46750=CARTESIAN_POINT ( 'NONE',  ( -5.481685914308793706, -284.4890048819452204, -337.4258668135261132 ) ) ;
#46751=CARTESIAN_POINT ( 'NONE',  ( -81.24783278021497779, -276.1412367623302657, -329.5469208930792888 ) ) ;
#46752=CARTESIAN_POINT ( 'NONE',  ( -6.411012262670094941, -275.5479530525081486, -203.8967017676368698 ) ) ;
#46754=CARTESIAN_POINT ( 'NONE',  ( -107.2764065286123127, -279.7641522453856169, -238.4006703163460941 ) ) ;
#46758=CARTESIAN_POINT ( 'NONE',  ( -94.89405966539744952, -287.0889195726613821, -221.0073457029371298 ) ) ;
#46759=CARTESIAN_POINT ( 'NONE',  ( 14.42332061702167501, -293.4986289255981546, -322.1332514729375589 ) ) ;
#46760=CARTESIAN_POINT ( 'NONE',  ( -113.5639656404338353, -290.0330084121748655, -259.7991293808597675 ) ) ;
#46761=CARTESIAN_POINT ( 'NONE',  ( 35.54144204940245544, -286.2611539220728218, -280.6223890411409911 ) ) ;
#46762=CARTESIAN_POINT ( 'NONE',  ( -108.7233414855515008, -289.0469154973205832, -250.8000522592148229 ) ) ;
#46763=CARTESIAN_POINT ( 'NONE',  ( -109.1050753979022545, -285.5544002912084238, -285.8203797214163160 ) ) ;
#46764=CARTESIAN_POINT ( 'NONE',  ( -110.7544795691030117, -276.7498517916012588, -254.9511784583348799 ) ) ;
#46765=CARTESIAN_POINT ( 'NONE',  ( 19.95773687891198378, -286.6389751872345641, -320.6123815290641232 ) ) ;
#46766=CARTESIAN_POINT ( 'NONE',  ( 36.80438653099493962, -289.4063156119605651, -258.9904778047576883 ) ) ;
#46767=CARTESIAN_POINT ( 'NONE',  ( 30.03257463744635558, -285.9920934755145367, -303.8061236370199367 ) ) ;
#46768=CARTESIAN_POINT ( 'NONE',  ( -33.47184316135159321, -283.9435351554913041, -343.5067102684656106 ) ) ;
#46769=CARTESIAN_POINT ( 'NONE',  ( -18.16683304624904594, -290.8057285031925403, -343.0409150103961906 ) ) ;
#46772=CARTESIAN_POINT ( 'NONE',  ( -110.8982473963231712, -298.2513033762172654, -287.7013503410714179 ) ) ;
#46773=CARTESIAN_POINT ( 'NONE',  ( 36.44873747522782281, -279.7251665673247771, -283.8483111841259756 ) ) ;
#46774=CARTESIAN_POINT ( 'NONE',  ( 24.69015057209802677, -292.1460437121533573, -225.0156847003438827 ) ) ;
#46775=CARTESIAN_POINT ( 'NONE',  ( -94.21720025602796511, -295.6116996783073319, -223.3136229615314789 ) ) ;
#46776=CARTESIAN_POINT ( 'NONE',  ( 30.48300365769452114, -279.8598692033370980, -242.0582376842496899 ) ) ;
#46777=CARTESIAN_POINT ( 'NONE',  ( 35.24324344331149916, -273.4176901811385960, -253.7891960201028496 ) ) ;
#46778=CARTESIAN_POINT ( 'NONE',  ( -78.21016175967831430, -296.9293425162473454, -331.5045904921583997 ) ) ;
#46780=CARTESIAN_POINT ( 'NONE',  ( -43.21688256451417232, -296.4592596781590714, -194.2282321944719001 ) ) ;
#46781=CARTESIAN_POINT ( 'NONE',  ( -41.90738058935478705, -293.3486667304447906, -346.2622022036466092 ) ) ;
#46782=CARTESIAN_POINT ( 'NONE',  ( 32.35327366383609160, -294.6642029286959996, -246.5808908674738689 ) ) ;
#46784=CARTESIAN_POINT ( 'NONE',  ( -3.570790652506796281, -293.3127541505124327, -205.4602135159243517 ) ) ;
#46786=CARTESIAN_POINT ( 'NONE',  ( -92.25068126354996423, -281.8523750196478090, -321.9882835814649980 ) ) ;
#46787=CARTESIAN_POINT ( 'NONE',  ( -7.988308176006066574, -294.6565936969429913, -337.2131452401724232 ) ) ;
#46788=CARTESIAN_POINT ( 'NONE',  ( -16.14183752788294512, -282.7855381839688107, -344.4404932703343434 ) ) ;
#46789=CARTESIAN_POINT ( 'NONE',  ( -4.309626302289554900, -282.4042502825120096, -202.3895616829989876 ) ) ;
#46790=CARTESIAN_POINT ( 'NONE',  ( -113.4658671525149316, -284.3663702048252730, -258.5705399046373714 ) ) ;
#46791=CARTESIAN_POINT ( 'NONE',  ( -109.8794375153375427, -288.7894100610452597, -251.9160026082831791 ) ) ;
#46793=CARTESIAN_POINT ( 'NONE',  ( -1.972848693455385272, -281.0722269068924106, -337.9758508630173424 ) ) ;
#46794=CARTESIAN_POINT ( 'NONE',  ( -29.02442258126227514, -287.8695485624459138, -346.6529711315224063 ) ) ;
#46796=CARTESIAN_POINT ( 'NONE',  ( 6.554967427744428754, -296.0447774294781880, -329.7503844756199101 ) ) ;
#46797=CARTESIAN_POINT ( 'NONE',  ( -51.18789780538250511, -278.6510966314526172, -345.5069036346620805 ) ) ;
#46798=CARTESIAN_POINT ( 'NONE',  ( -34.30820238962408553, -279.7580201447307786, -197.3904638657029693 ) ) ;
#46799=CARTESIAN_POINT ( 'NONE',  ( -25.02353168793252536, -292.3717848219060897, -194.3528109972795619 ) ) ;
#46800=CARTESIAN_POINT ( 'NONE',  ( -112.0596581951970450, -282.7797534199804090, -258.7677926004978417 ) ) ;
#46801=CARTESIAN_POINT ( 'NONE',  ( -94.60523539357275524, -279.8821134007427531, -318.8153014472902100 ) ) ;
#46803=CARTESIAN_POINT ( 'NONE',  ( -2.316393565318947356, -291.5864189557678401, -206.0301879968598087 ) ) ;
#46804=CARTESIAN_POINT ( 'NONE',  ( -111.6174256862581586, -294.6866888243472999, -259.8704963559827661 ) ) ;
#46807=CARTESIAN_POINT ( 'NONE',  ( -5.520368767034310231, -294.1295451126133003, -336.1426467329376351 ) ) ;
#46810=CARTESIAN_POINT ( 'NONE',  ( -6.998514795304330072, -292.1237833571632336, -333.4427485647536855 ) ) ;
#46811=CARTESIAN_POINT ( 'NONE',  ( -112.9075915997575663, -271.9274202390725463, -256.1504789243317646 ) ) ;
#46812=CARTESIAN_POINT ( 'NONE',  ( 26.71564516297948089, -288.3141868991640990, -228.5286570616940764 ) ) ;
#46813=CARTESIAN_POINT ( 'NONE',  ( 19.51214923481084895, -288.0328525565698783, -316.1501976540363898 ) ) ;
#46814=CARTESIAN_POINT ( 'NONE',  ( -70.74998003744313735, -279.0212814498722764, -336.0466916479080624 ) ) ;
#46815=CARTESIAN_POINT ( 'NONE',  ( -35.81142357793161324, -299.8317057372617569, -196.3473114662746184 ) ) ;
#46816=CARTESIAN_POINT ( 'NONE',  ( -87.37737015061139800, -276.5639099852722893, -324.0599282993237011 ) ) ;
#46818=CARTESIAN_POINT ( 'NONE',  ( -113.0678965813541197, -272.5634699782864914, -256.1286169489388271 ) ) ;
#46819=CARTESIAN_POINT ( 'NONE',  ( -109.5104580981725206, -292.7090905254490849, -252.0613424212702114 ) ) ;
#46820=CARTESIAN_POINT ( 'NONE',  ( 24.15662711807824081, -294.5486163513410816, -225.3678277859163472 ) ) ;
#46822=CARTESIAN_POINT ( 'NONE',  ( -88.72683398023475831, -290.4486016215405471, -322.3559320226291902 ) ) ;
#46825=CARTESIAN_POINT ( 'NONE',  ( 1.094246314520575192, -290.6986517721620089, -205.0096254285737700 ) ) ;
#46826=CARTESIAN_POINT ( 'NONE',  ( -33.34011082396492753, -298.4342490044799092, -193.3820424796144266 ) ) ;
#46827=CARTESIAN_POINT ( 'NONE',  ( -40.51464284768410096, -297.6779089888000840, -197.3963899822251449 ) ) ;
#46830=CARTESIAN_POINT ( 'NONE',  ( -82.42726890285256047, -291.1755718613267732, -331.9240876904858624 ) ) ;
#46831=CARTESIAN_POINT ( 'NONE',  ( -115.3288506153726871, -286.8376638359844719, -288.1938231032136741 ) ) ;
#46832=CARTESIAN_POINT ( 'NONE',  ( -65.81377399587834987, -287.6791493850333836, -201.1006789375407777 ) ) ;
#46833=CARTESIAN_POINT ( 'NONE',  ( -36.69527521088521382, -272.0601337886153601, -195.5178449881298377 ) ) ;
#46834=CARTESIAN_POINT ( 'NONE',  ( 36.53832420928921465, -277.5955393794843076, -279.8868183234383196 ) ) ;
#46835=CARTESIAN_POINT ( 'NONE',  ( -64.57611798041747875, -289.7736945246065261, -201.0681696380719927 ) ) ;
#46836=CARTESIAN_POINT ( 'NONE',  ( -45.49279707765411729, -279.0146684454041974, -345.7383876816082307 ) ) ;
#46838=CARTESIAN_POINT ( 'NONE',  ( -34.85136655472116018, -282.3686655291266447, -343.4330745383493877 ) ) ;
#46839=CARTESIAN_POINT ( 'NONE',  ( -107.1435071399293406, -280.0409465176456365, -238.4652964810486822 ) ) ;
#46840=CARTESIAN_POINT ( 'NONE',  ( 35.80115906322091490, -280.0596480845708811, -247.5986298077007746 ) ) ;
#46841=CARTESIAN_POINT ( 'NONE',  ( 197.4573848121495416, 287.6755661058302849, -96.60709594317813753 ) ) ;
#46842=CARTESIAN_POINT ( 'NONE',  ( 21.55782282952521101, -277.1579230107995500, -319.5918645658061337 ) ) ;
#46845=B_SPLINE_CURVE_WITH_KNOTS ( 'NONE', 3,
 ( #20345, #92760, #13252, #49677, #29314, #56817, #72406, #85659, #86578, #63454, #19862, #41628, #48733, #35946, #64405, #57277, #27440, #14190, #70548, #42561, #71478, #5671, #86119, #34546, #57732, #79038, #21747, #79514 ),
 .UNSPECIFIED., .F., .F.,
 ( 4, 2, 2, 2, 2, 2, 2, 2, 2, 2, 2, 2, 2, 4 ),
 ( 0.007868691692155720466, 0.008845612455071254210, 0.009334072836528988990, 0.009822533217986722034, 0.01031099359944445681, 0.01079945398090218986, 0.01128791436235992290, 0.01177637474381765595, 0.01226483512527539073, 0.01275329550673312551, 0.01324175588819085855, 0.01373021626964859160, 0.01470713703256412014, 0.01568405779547964868 ),
 .UNSPECIFIED. ) ;
#46846=CARTESIAN_POINT ( 'NONE',  ( 2.043418945047154711, -276.0894731127471573, -205.0042503412220753 ) ) ;
#46847=CARTESIAN_POINT ( 'NONE',  ( 21.31550574532285580, -296.6948066931273615, -317.0979686699210447 ) ) ;
#46851=CARTESIAN_POINT ( 'NONE',  ( -42.67272446439136502, -290.2005196228595310, -343.5269567670270021 ) ) ;
#46852=CARTESIAN_POINT ( 'NONE',  ( 31.78079137556968092, -288.9019993375378021, -238.6741920333060420 ) ) ;
#46853=CARTESIAN_POINT ( 'NONE',  ( -107.0963991988017767, -290.1906483991432424, -248.4517607941682513 ) ) ;
#46854=CARTESIAN_POINT ( 'NONE',  ( -57.73358334943154091, -285.3034630765065458, -196.1188992306328203 ) ) ;
#46856=CARTESIAN_POINT ( 'NONE',  ( 36.48818723402094832, -279.9288325332478280, -268.5844290499083513 ) ) ;
#46857=CARTESIAN_POINT ( 'NONE',  ( 14.97032150275138562, -290.1651754952927718, -323.0329118777052599 ) ) ;
#46858=CARTESIAN_POINT ( 'NONE',  ( -37.56185159518126682, -281.5348691761150235, -344.0666728013138709 ) ) ;
#46859=CARTESIAN_POINT ( 'NONE',  ( -81.59810958637109479, -280.7509618162966945, -211.6234148026327944 ) ) ;
#46860=CARTESIAN_POINT ( 'NONE',  ( 37.14560079645574575, -288.2604895310776101, -251.8014246977716084 ) ) ;
#46861=CARTESIAN_POINT ( 'NONE',  ( -103.1837504123561615, -278.6150238893242772, -302.1453812113981030 ) ) ;
#46862=CARTESIAN_POINT ( 'NONE',  ( -98.87641883833006773, -289.9570058609152738, -224.7158321821602271 ) ) ;
#46863=CARTESIAN_POINT ( 'NONE',  ( -54.93758100951860968, -286.6342948651698066, -195.5644349277536946 ) ) ;
#46864=CARTESIAN_POINT ( 'NONE',  ( -73.58957004187121242, -286.0769947834070877, -202.4373991479402832 ) ) ;
#46865=CARTESIAN_POINT ( 'NONE',  ( -65.31373319830633761, -283.5948945566061070, -337.8029401839038997 ) ) ;
#46868=CARTESIAN_POINT ( 'NONE',  ( -69.12693003084130794, -293.4989792609995334, -201.5719757696961096 ) ) ;
#46869=CARTESIAN_POINT ( 'NONE',  ( 30.46963714374363263, -291.7757163938274516, -234.8221605571063435 ) ) ;
#46870=CARTESIAN_POINT ( 'NONE',  ( 35.33806040673717064, -274.7345947034932578, -279.7684096025811868 ) ) ;
#46871=CARTESIAN_POINT ( 'NONE',  ( -109.3450226567610883, -295.5571032897107102, -297.5083259787439260 ) ) ;
#46873=CARTESIAN_POINT ( 'NONE',  ( -66.82384580459678602, -290.1385310595077272, -202.8221600386912939 ) ) ;
#46874=CARTESIAN_POINT ( 'NONE',  ( -47.96027363389119813, -293.4287651625002695, -343.6607731370596639 ) ) ;
#46875=CARTESIAN_POINT ( 'NONE',  ( -81.98264858339445027, -292.6335779687863123, -212.0360335224583821 ) ) ;
#46877=CARTESIAN_POINT ( 'NONE',  ( 14.20003917586191555, -290.7735027746303444, -215.5769466340024678 ) ) ;
#46879=CARTESIAN_POINT ( 'NONE',  ( 33.08241283956743217, -295.2159507105831153, -244.4172390993785768 ) ) ;
#46880=CARTESIAN_POINT ( 'NONE',  ( 19.70428784401630651, -289.1406051773078616, -316.2867503160322258 ) ) ;
#46881=CARTESIAN_POINT ( 'NONE',  ( -39.88170544273447859, -279.0637725825090456, -345.6862893238195511 ) ) ;
#46882=CARTESIAN_POINT ( 'NONE',  ( -104.6341327016061484, -276.8709806574642585, -306.9635391579996053 ) ) ;
#46883=CARTESIAN_POINT ( 'NONE',  ( -75.69042796910599691, -296.7514776721768612, -203.7152706514069109 ) ) ;
#46884=CARTESIAN_POINT ( 'NONE',  ( -7.114024572189377338, -274.8898898864312059, -337.9204374448056001 ) ) ;
#46885=CARTESIAN_POINT ( 'NONE',  ( -95.90894070865891763, -277.2675540450228482, -224.3928957015725132 ) ) ;
#46886=CARTESIAN_POINT ( 'NONE',  ( -59.45254646894837691, -275.7336684753215650, -343.2826572415415285 ) ) ;
#46887=CARTESIAN_POINT ( 'NONE',  ( -110.7035680661494297, -295.2945055766592191, -265.9702399943167848 ) ) ;
#46889=CARTESIAN_POINT ( 'NONE',  ( -83.26104478151587784, -274.0549525008167393, -213.4813636368857317 ) ) ;
#46891=CARTESIAN_POINT ( 'NONE',  ( -54.15959457129459764, -287.2870430271519240, -343.8691761463691705 ) ) ;
#46892=CARTESIAN_POINT ( 'NONE',  ( 34.84197555492129084, -275.2407499413783967, -259.3904458100947750 ) ) ;
#46893=CARTESIAN_POINT ( 'NONE',  ( 38.02350660930691362, -287.3539724695729092, -254.5148300327509503 ) ) ;
#46894=CARTESIAN_POINT ( 'NONE',  ( -88.92373787837848909, -275.3300913450562462, -215.6153242181658527 ) ) ;
#46895=CARTESIAN_POINT ( 'NONE',  ( -99.96823353129545353, -295.1069028351938073, -229.3046556303672503 ) ) ;
#46896=CARTESIAN_POINT ( 'NONE',  ( -90.33419302872037804, -282.9760711694154338, -326.0753856950369709 ) ) ;
#46898=CARTESIAN_POINT ( 'NONE',  ( 21.47023816398901630, -278.9124881820549149, -223.7988820376661749 ) ) ;
#46900=CARTESIAN_POINT ( 'NONE',  ( -109.5723982504696750, -289.1760770719048423, -283.3940284143973258 ) ) ;
#46903=CARTESIAN_POINT ( 'NONE',  ( -66.07012327224013859, -289.6760666312246144, -201.0675250192834937 ) ) ;
#46904=CARTESIAN_POINT ( 'NONE',  ( -34.02869719533108395, -275.6147018488665594, -196.7422904642450305 ) ) ;
#46905=CARTESIAN_POINT ( 'NONE',  ( 38.20931589831229047, -282.8290493070682601, -258.5882457565131176 ) ) ;
#46906=CARTESIAN_POINT ( 'NONE',  ( -95.80601951000305405, -271.2871524245595083, -222.4740616317136528 ) ) ;
#46907=CARTESIAN_POINT ( 'NONE',  ( -53.68966852611506368, -283.2676916330322001, -341.5591363401455283 ) ) ;
#46908=CARTESIAN_POINT ( 'NONE',  ( -2.651801216718761456, -275.9456819964217402, -205.4613041789028216 ) ) ;
#46909=CARTESIAN_POINT ( 'NONE',  ( 33.01247274742645033, -276.0880278155352698, -250.1080145665276575 ) ) ;
#46911=CARTESIAN_POINT ( 'NONE',  ( -70.82245150820266133, -285.4939989542326089, -337.4732624858654049 ) ) ;
#46912=CARTESIAN_POINT ( 'NONE',  ( -83.37405570498910379, -272.3241464575996247, -213.3063345488225764 ) ) ;
#46915=CARTESIAN_POINT ( 'NONE',  ( 35.48572158426885892, -293.7024345034074599, -295.5278303757756930 ) ) ;
#46916=CARTESIAN_POINT ( 'NONE',  ( -109.3411367842514750, -286.2769992143743707, -290.1052003954233101 ) ) ;
#46918=CARTESIAN_POINT ( 'NONE',  ( -99.86837403722181250, -276.6952119285918457, -220.4570493818173702 ) ) ;
#46919=CARTESIAN_POINT ( 'NONE',  ( -34.30772645810454691, -276.2120856266992632, -347.1397206309391095 ) ) ;
#46920=CARTESIAN_POINT ( 'NONE',  ( -94.86788344615027313, -288.2695244997815962, -320.3328965143486471 ) ) ;
#46921=CARTESIAN_POINT ( 'NONE',  ( -68.05585817551738614, -284.9830711392421563, -337.3487903542435333 ) ) ;
#46922=CARTESIAN_POINT ( 'NONE',  ( -51.45242795770836608, -278.9952236349207624, -343.0168911265149063 ) ) ;
#46923=CARTESIAN_POINT ( 'NONE',  ( -85.15841457249160840, -286.8317358163424728, -210.7610499371244543 ) ) ;
#46924=CARTESIAN_POINT ( 'NONE',  ( 33.86769820320593283, -283.2462194376556681, -246.6556805340865708 ) ) ;
#46925=CARTESIAN_POINT ( 'NONE',  ( -55.33567763507367232, -273.9935013321080532, -195.4931222970732279 ) ) ;
#46926=CARTESIAN_POINT ( 'NONE',  ( -113.0660165063659122, -278.2100017788474702, -284.3916475938056578 ) ) ;
#46927=CARTESIAN_POINT ( 'NONE',  ( -78.73047227620422461, -297.5342251296269183, -332.2964913152691793 ) ) ;
#46929=CARTESIAN_POINT ( 'NONE',  ( -110.4542110544635705, -280.8376638359844719, -287.0812184334320705 ) ) ;
#46930=CARTESIAN_POINT ( 'NONE',  ( -62.41359801023755693, -295.8689833392643322, -198.8649263636822866 ) ) ;
#46931=CARTESIAN_POINT ( 'NONE',  ( -43.21828445101425586, -276.6360115185968311, -343.1859365431740230 ) ) ;
#46932=CARTESIAN_POINT ( 'NONE',  ( -35.54854423031162725, -275.2792216778477155, -193.7661167871499401 ) ) ;
#46934=CARTESIAN_POINT ( 'NONE',  ( 29.71876917803477269, -288.8951686610731713, -239.0423142484046366 ) ) ;
#46935=CARTESIAN_POINT ( 'NONE',  ( -64.00561790569661014, -296.9138414628872624, -341.8575741261659005 ) ) ;
#46936=CARTESIAN_POINT ( 'NONE',  ( -41.90647906290507763, -296.3134049404910684, -346.8800417321108966 ) ) ;
#46937=CARTESIAN_POINT ( 'NONE',  ( 32.53132825814162032, -295.2032517806943019, -243.5695460121583267 ) ) ;
#46938=CARTESIAN_POINT ( 'NONE',  ( -39.73497317003972995, -278.0218940957681184, -195.5532257248924566 ) ) ;
#46939=CARTESIAN_POINT ( 'NONE',  ( 36.12867188484763403, -283.6272326712789322, -282.3368699507942097 ) ) ;
#46940=CARTESIAN_POINT ( 'NONE',  ( -67.37839407562766780, -295.7349918527977479, -202.2361494568315550 ) ) ;
#46941=CARTESIAN_POINT ( 'NONE',  ( -49.86561904497637698, -285.0705581024865864, -345.1366598365087839 ) ) ;
#46942=CARTESIAN_POINT ( 'NONE',  ( -9.362743454458945180, -285.3469755665719276, -202.5876515215307450 ) ) ;
#46943=CARTESIAN_POINT ( 'NONE',  ( 169.6770662837093084, 231.1674941253104976, -192.2518117328845904 ) ) ;
#46945=CARTESIAN_POINT ( 'NONE',  ( 16.90916867492576614, -286.5190481281735515, -221.4657607458265716 ) ) ;
#46947=CARTESIAN_POINT ( 'NONE',  ( -106.7201388501397901, -285.2114947837844738, -303.0432958377926980 ) ) ;
#46948=CARTESIAN_POINT ( 'NONE',  ( -107.2180051618227310, -273.1681140090341273, -248.9890690553962997 ) ) ;
#46949=CARTESIAN_POINT ( 'NONE',  ( 28.36588968391163235, -285.8297558394187377, -230.8821231114277737 ) ) ;
#46950=CARTESIAN_POINT ( 'NONE',  ( -102.9442683331660504, -289.9941773925558550, -230.5372848800695067 ) ) ;
#46951=CARTESIAN_POINT ( 'NONE',  ( 17.04791332139559401, -281.7454161081065536, -216.1147364500776007 ) ) ;
#46953=CARTESIAN_POINT ( 'NONE',  ( -112.0428259243559239, -280.2695635856457557, -254.7272348855554753 ) ) ;
#46954=CARTESIAN_POINT ( 'NONE',  ( 38.77316867427907709, -281.7372344245923728, -258.5146077812706835 ) ) ;
#46955=CARTESIAN_POINT ( 'NONE',  ( 7.399455738971487229, -285.9094976428776249, -326.5171145203363494 ) ) ;
#46956=CARTESIAN_POINT ( 'NONE',  ( 194.8177507750399400, 278.8342080080603864, -125.9237472059935925 ) ) ;
#46958=CARTESIAN_POINT ( 'NONE',  ( 19.72253917211401131, -278.2237576157742751, -318.7729039706862295 ) ) ;
#46959=CARTESIAN_POINT ( 'NONE',  ( -40.44464271085224993, -139.2070877199659549, -364.2637007583950890 ) ) ;
#46960=CARTESIAN_POINT ( 'NONE',  ( 3.627343256310792352, -278.6259450273276457, -207.9020939042410134 ) ) ;
#46961=CARTESIAN_POINT ( 'NONE',  ( 20.60956065430444539, -295.9835890928820277, -319.5101300760515528 ) ) ;
#46962=CARTESIAN_POINT ( 'NONE',  ( -84.55024615857061576, -295.0708339854741666, -326.2419744307011911 ) ) ;
#46963=CARTESIAN_POINT ( 'NONE',  ( -105.9463953377612597, -290.5098734150645328, -235.4166268970972453 ) ) ;
#46965=CARTESIAN_POINT ( 'NONE',  ( -110.2454253371586503, -295.4186315915780483, -247.3023882779304756 ) ) ;
#46966=CARTESIAN_POINT ( 'NONE',  ( 1.717907479817098571, -286.9201072494794857, -332.9773097230851135 ) ) ;
#46967=CARTESIAN_POINT ( 'NONE',  ( 29.84655285367539435, -294.9917865583138337, -238.6708420628921488 ) ) ;
#46968=CARTESIAN_POINT ( 'NONE',  ( 7.212683526540816459, -287.9886006751912646, -211.8489868194129997 ) ) ;
#46969=VERTEX_POINT ( 'NONE', #47603 ) ;
#46970=CARTESIAN_POINT ( 'NONE',  ( -8.610440935211915559, -293.3603645007340788, -199.1759021136741694 ) ) ;
#46971=CARTESIAN_POINT ( 'NONE',  ( -105.2688351451556343, -284.6832523746464290, -297.4040598760556122 ) ) ;
#46972=CARTESIAN_POINT ( 'NONE',  ( -96.21614267100038376, -294.6843027927102980, -319.3897710384776474 ) ) ;
#46973=CARTESIAN_POINT ( 'NONE',  ( -107.5796045707633937, -290.9550515346834914, -301.6495358087673822 ) ) ;
#46975=CARTESIAN_POINT ( 'NONE',  ( -92.77210578817116016, -291.7761981067884562, -216.9280578369938723 ) ) ;
#46976=CARTESIAN_POINT ( 'NONE',  ( -100.3028759983042448, -290.2103514610667503, -307.4050967936290135 ) ) ;
#46979=CARTESIAN_POINT ( 'NONE',  ( -90.78135383411671455, -299.1642829180493095, -216.6534938395993777 ) ) ;
#46980=CARTESIAN_POINT ( 'NONE',  ( -113.4663574789698117, -271.4545208574642174, -261.8144659321022232 ) ) ;
#46982=CARTESIAN_POINT ( 'NONE',  ( -24.03446288130383834, -281.9367339217170070, -342.3772681456105147 ) ) ;
#46983=CARTESIAN_POINT ( 'NONE',  ( 13.92814348106507438, -274.2561390963737153, -212.9232892548436951 ) ) ;
#46984=CARTESIAN_POINT ( 'NONE',  ( -107.5355677566599013, -294.7353018575846022, -292.9658994180929881 ) ) ;
#46985=CARTESIAN_POINT ( 'NONE',  ( -41.90930862228105980, -278.9707065260643049, -344.4684782110286960 ) ) ;
#46986=CARTESIAN_POINT ( 'NONE',  ( -33.96111872393461795, -272.2347102126651066, -196.2029279331675582 ) ) ;
#46987=CARTESIAN_POINT ( 'NONE',  ( -52.73325169411006641, -299.0557440639112201, -198.5438408901347600 ) ) ;
#46988=CARTESIAN_POINT ( 'NONE',  ( -108.7813540979411471, -297.8479139283605832, -253.9111357514047711 ) ) ;
#46990=CARTESIAN_POINT ( 'NONE',  ( -70.40059192125617926, -299.2237437361544039, -201.7058188978544422 ) ) ;
#46991=CARTESIAN_POINT ( 'NONE',  ( -106.5565295716641430, -270.9616159465771830, -240.4347256797260854 ) ) ;
#46992=CARTESIAN_POINT ( 'NONE',  ( 8.298268712311218209, -295.0602075196611054, -327.5303473707286912 ) ) ;
#46993=CARTESIAN_POINT ( 'NONE',  ( 0.2253321349396642526, -291.1377977693260277, -207.0832150137832741 ) ) ;
#46995=CARTESIAN_POINT ( 'NONE',  ( 38.15715175967597617, -275.8590810657676684, -255.5472640931754711 ) ) ;
#46996=CARTESIAN_POINT ( 'NONE',  ( -91.12397300751980822, -273.4274203740927760, -220.9820303778206494 ) ) ;
#46997=CARTESIAN_POINT ( 'NONE',  ( 36.63506767828697974, -283.3486921252967932, -256.0138314624815621 ) ) ;
#46998=CARTESIAN_POINT ( 'NONE',  ( -50.02833169424848592, -281.8954793530547818, -345.8622978835057893 ) ) ;
#46999=CARTESIAN_POINT ( 'NONE',  ( -100.3866959098494505, -277.3179440326601366, -314.3911224516833158 ) ) ;
#47001=CARTESIAN_POINT ( 'NONE',  ( -107.5069076522069764, -284.0250114670508879, -249.4624343582494532 ) ) ;
#47002=CARTESIAN_POINT ( 'NONE',  ( -93.97073002194308344, -281.8672429092375751, -319.7896664334157322 ) ) ;
#47003=CARTESIAN_POINT ( 'NONE',  ( 21.29552399324870038, -274.7467529015071932, -314.8251581273250963 ) ) ;
#47004=CARTESIAN_POINT ( 'NONE',  ( -67.15354586629744915, -281.6616284565767501, -201.4860309758704773 ) ) ;
#47006=DIRECTION ( 'NONE',  ( 1.000000000000000000, 0.000000000000000000, 0.000000000000000000 ) ) ;
#47007=CARTESIAN_POINT ( 'NONE',  ( -38.32642062593526333, -272.4398796970623380, -194.1674781969756509 ) ) ;
#47009=CARTESIAN_POINT ( 'NONE',  ( -111.4337740989455057, -280.7145634918160226, -257.6964820701455210 ) ) ;
#47011=CARTESIAN_POINT ( 'NONE',  ( -112.7173390553466419, -286.5484470036557241, -264.3869059452312058 ) ) ;
#47013=CARTESIAN_POINT ( 'NONE',  ( 37.47891543908901468, -285.4765352301147914, -264.4846717265897382 ) ) ;
#47015=CARTESIAN_POINT ( 'NONE',  ( -100.5160206574300190, -294.8352570375583923, -307.8261266774889577 ) ) ;
#47016=CARTESIAN_POINT ( 'NONE',  ( -61.68200203203052467, -287.5114067677779417, -340.4925316464137950 ) ) ;
#47017=CARTESIAN_POINT ( 'NONE',  ( -90.78337343436103879, -230.3218577325732781, -348.1307343985224634 ) ) ;
#47018=CARTESIAN_POINT ( 'NONE',  ( -83.14596724027933305, -295.4252801002794513, -210.9070174246385818 ) ) ;
#47019=CARTESIAN_POINT ( 'NONE',  ( -46.40378332877921252, -284.4190197345153592, -194.5944604093216128 ) ) ;
#47020=CARTESIAN_POINT ( 'NONE',  ( 19.43869558214458237, -282.4907071640962499, -223.1988870093859703 ) ) ;
#47021=CARTESIAN_POINT ( 'NONE',  ( -19.18257339715441034, -281.0615910928992207, -344.2003073555125638 ) ) ;
#47022=CARTESIAN_POINT ( 'NONE',  ( 1.311582375930386180, -288.5199776905834028, -332.2878791740275801 ) ) ;
#47023=CARTESIAN_POINT ( 'NONE',  ( -71.22902915375870236, -281.0209491235688120, -205.0244547385905776 ) ) ;
#47024=CARTESIAN_POINT ( 'NONE',  ( -46.48675635365798797, -280.7361043481161005, -197.7222332245394796 ) ) ;
#47025=CARTESIAN_POINT ( 'NONE',  ( 37.15559972513672449, -289.3860505917339196, -258.9370011673490239 ) ) ;
#47026=VERTEX_POINT ( 'NONE', #70358 ) ;
#47027=CARTESIAN_POINT ( 'NONE',  ( -60.87111981962079454, -273.7551671876918249, -196.9885975298930418 ) ) ;
#47028=CARTESIAN_POINT ( 'NONE',  ( -108.9808215216218059, -292.8038699917130430, -249.3470570570178495 ) ) ;
#47030=CARTESIAN_POINT ( 'NONE',  ( 39.58706461736021254, -290.0519495502703080, -270.3284710469133074 ) ) ;
#47033=CARTESIAN_POINT ( 'NONE',  ( 18.49778037380008300, -274.2519160745908380, -320.6991646455864498 ) ) ;
#47036=CARTESIAN_POINT ( 'NONE',  ( -85.90133934816454087, -294.1119703109618513, -329.0842126918170152 ) ) ;
#47037=CARTESIAN_POINT ( 'NONE',  ( -81.12543524878962842, -272.7882670244369478, -211.7580701082218582 ) ) ;
#47038=CARTESIAN_POINT ( 'NONE',  ( -108.3891023910953919, -291.8139158061215426, -290.1187138804352799 ) ) ;
#47039=CARTESIAN_POINT ( 'NONE',  ( -45.73239137491702877, -284.9199658065680865, -343.9490024771080243 ) ) ;
#47040=CARTESIAN_POINT ( 'NONE',  ( -111.6851506909061129, -291.7542241589767400, -288.0708758724734366 ) ) ;
#47041=CARTESIAN_POINT ( 'NONE',  ( -109.0177512386438963, -292.2095821832967317, -243.4548305301497919 ) ) ;
#47042=CARTESIAN_POINT ( 'NONE',  ( 17.07915138694823654, -294.0816774226379380, -319.0355997970497697 ) ) ;
#47043=CARTESIAN_POINT ( 'NONE',  ( -30.37006322470126918, -288.1403637804345408, -195.6336520173842075 ) ) ;
#47044=CARTESIAN_POINT ( 'NONE',  ( 4.547477976340775108, -282.6706721715551112, -335.0329348870571948 ) ) ;
#47045=CARTESIAN_POINT ( 'NONE',  ( -108.4866263536419808, -294.9593919667693172, -244.9108985521590114 ) ) ;
#47046=CARTESIAN_POINT ( 'NONE',  ( -61.23368828972838429, -283.1872046948417392, -343.6163446926947245 ) ) ;
#47047=CARTESIAN_POINT ( 'NONE',  ( 20.47116220953870780, -278.1860270779059192, -317.5990592484021136 ) ) ;
#47048=CARTESIAN_POINT ( 'NONE',  ( -92.08974858914540107, -293.6948066931273047, -226.7417163044926838 ) ) ;
#47049=CARTESIAN_POINT ( 'NONE',  ( -112.9998279212854015, -276.6406517938480079, -274.3802194925361846 ) ) ;
#47051=CARTESIAN_POINT ( 'NONE',  ( -34.85071812533317370, -282.5277058291583216, -343.3926273606829227 ) ) ;
#47052=CARTESIAN_POINT ( 'NONE',  ( -104.4531380688512030, -280.2380577036137765, -233.4278861294972103 ) ) ;
#47053=CARTESIAN_POINT ( 'NONE',  ( 2.628757674676041933, -285.6331815795425655, -204.8234744806161700 ) ) ;
#47054=CARTESIAN_POINT ( 'NONE',  ( -5.627472017059326426, -294.2352124802760045, -203.4727743469865118 ) ) ;
#47055=CARTESIAN_POINT ( 'NONE',  ( 0.7773851988820995595, -276.1517640811136971, -204.3658774473878168 ) ) ;
#47056=CARTESIAN_POINT ( 'NONE',  ( 17.72294824480497866, -276.1346321005822233, -217.1702791299086073 ) ) ;
#47057=CARTESIAN_POINT ( 'NONE',  ( -37.81189010033128284, -276.8914866397913102, -343.3720566061695649 ) ) ;
#47058=CARTESIAN_POINT ( 'NONE',  ( -68.84189627889301732, -299.6372711097631623, -202.4665806840606876 ) ) ;
#47059=CARTESIAN_POINT ( 'NONE',  ( -101.1598074412561346, -283.0784820371161459, -231.1820421061018180 ) ) ;
#47060=CARTESIAN_POINT ( 'NONE',  ( 33.30667356818824487, -292.8292079152202518, -239.7906815199799269 ) ) ;
#47061=CARTESIAN_POINT ( 'NONE',  ( -105.7858829580553959, -291.7162770810338088, -303.9747858199236248 ) ) ;
#47062=CARTESIAN_POINT ( 'NONE',  ( -3.481310526433006203, -291.4305545795600096, -205.3403513735555919 ) ) ;
#47064=CARTESIAN_POINT ( 'NONE',  ( -37.77334838268598105, -290.6215795207753558, -193.9515637679012059 ) ) ;
#47065=CARTESIAN_POINT ( 'NONE',  ( -6.028715400097473420, -292.1421290203160197, -204.3807910971478918 ) ) ;
#47066=ORIENTED_EDGE ( 'NONE', *, *, #73502, .T. ) ;
#47067=CARTESIAN_POINT ( 'NONE',  ( -73.01782587618470188, -290.5933111271570510, -338.2632691896680512 ) ) ;
#47068=CARTESIAN_POINT ( 'NONE',  ( -108.0733132660293876, -279.4475922210236263, -251.8475943923816374 ) ) ;
#47069=CARTESIAN_POINT ( 'NONE',  ( -57.29598324438435952, -296.7209759230235022, -196.2566271848827739 ) ) ;
#47070=CARTESIAN_POINT ( 'NONE',  ( -68.46711259473553923, -286.3052545824558592, -200.0294683858754183 ) ) ;
#47071=CARTESIAN_POINT ( 'NONE',  ( 34.83293126133888507, -287.5469013258806967, -243.5923511961041754 ) ) ;
#47072=CARTESIAN_POINT ( 'NONE',  ( -108.6864749445183946, -285.0913634823190250, -254.7460366052251572 ) ) ;
#47073=CARTESIAN_POINT ( 'NONE',  ( -114.0438498157189002, -273.6021558389782058, -270.3744870444270418 ) ) ;
#47074=CARTESIAN_POINT ( 'NONE',  ( -64.84513123375332100, -181.9241928666178012, -360.8394250873944884 ) ) ;
#47075=CARTESIAN_POINT ( 'NONE',  ( -48.11459895883137960, -154.8715929890281018, -361.3444938967305120 ) ) ;
#47077=CARTESIAN_POINT ( 'NONE',  ( 35.54004119667265371, -274.6578938696477508, -263.4155625949403543 ) ) ;
#47078=CARTESIAN_POINT ( 'NONE',  ( 24.23659503619849431, -275.0219747546571512, -310.2333248977112703 ) ) ;
#47079=CARTESIAN_POINT ( 'NONE',  ( -102.2611045658888997, -296.6014632875123311, -229.0694986076424016 ) ) ;
#47080=CARTESIAN_POINT ( 'NONE',  ( 194.3800462488992764, 275.6740546377429837, -124.2862691682898912 ) ) ;
#47081=CARTESIAN_POINT ( 'NONE',  ( 15.69729037477889477, -273.4690764703283321, -215.2234379593620872 ) ) ;
#47082=CARTESIAN_POINT ( 'NONE',  ( -62.39347726987958254, -275.4818730019001691, -200.7164306406782259 ) ) ;
#47084=CARTESIAN_POINT ( 'NONE',  ( -112.1448397258379259, -273.8441659360954645, -253.4500914685297630 ) ) ;
#47086=CARTESIAN_POINT ( 'NONE',  ( -86.76639950507839671, -290.2539334107912623, -324.2366916710582814 ) ) ;
#47087=CARTESIAN_POINT ( 'NONE',  ( -113.4911810375529058, -297.2214278826049281, -281.0176193153636746 ) ) ;
#47088=CARTESIAN_POINT ( 'NONE',  ( -87.42695835512067504, -297.8678430461726521, -211.8871664294761956 ) ) ;
#47089=CARTESIAN_POINT ( 'NONE',  ( -31.60023773765314914, -295.1444758661645551, -343.1850974472641838 ) ) ;
#47091=CARTESIAN_POINT ( 'NONE',  ( 2.758408817152785630, -278.4392578322497229, -334.4640773364017150 ) ) ;
#47092=CARTESIAN_POINT ( 'NONE',  ( -6.249483265708501101, -279.9574497234660839, -199.9707174285328506 ) ) ;
#47093=CARTESIAN_POINT ( 'NONE',  ( -87.24714235409743424, -278.7098920521756895, -323.9601411440245329 ) ) ;
#47094=CARTESIAN_POINT ( 'NONE',  ( 2.982998827523904772, -278.2792707822525813, -334.8272022141157436 ) ) ;
#47095=CARTESIAN_POINT ( 'NONE',  ( -94.66489187455550791, -273.6831936119405668, -225.0616684287499254 ) ) ;
#47096=CARTESIAN_POINT ( 'NONE',  ( -73.11759151502221243, -296.1426784653517075, -206.0535716657066416 ) ) ;
#47098=CARTESIAN_POINT ( 'NONE',  ( -110.1587953022172712, -278.7869597853193682, -265.1967540440379025 ) ) ;
#47099=CARTESIAN_POINT ( 'NONE',  ( 15.90775751242345670, -275.5867418297112295, -214.9656842252709623 ) ) ;
#47100=CARTESIAN_POINT ( 'NONE',  ( 19.24812447804917781, -286.9414441284055215, -321.8674212866099538 ) ) ;
#47101=CARTESIAN_POINT ( 'NONE',  ( -41.11822994884737170, -276.0049114319845103, -195.4053537863085808 ) ) ;
#47103=CARTESIAN_POINT ( 'NONE',  ( -108.8226826575141928, -289.5433933827991950, -286.0101253852195669 ) ) ;
#47104=CARTESIAN_POINT ( 'NONE',  ( -103.9480126313587647, -284.4022051548209902, -231.8246337239282013 ) ) ;
#47105=CARTESIAN_POINT ( 'NONE',  ( 29.90259401685330332, -279.3791176051769298, -239.3160701446660994 ) ) ;
#47106=CARTESIAN_POINT ( 'NONE',  ( 30.57220201244553337, -279.7497886464838643, -242.0225080704779828 ) ) ;
#47107=CARTESIAN_POINT ( 'NONE',  ( -55.07615895754810253, -283.9023055931288013, -198.0111594346907395 ) ) ;
#47108=CARTESIAN_POINT ( 'NONE',  ( -4.615593536979407219, -290.6212791180838053, -337.8584503209099807 ) ) ;
#47109=CARTESIAN_POINT ( 'NONE',  ( -108.9977426909084528, -279.9664205971453157, -254.4119552648612625 ) ) ;
#47111=CARTESIAN_POINT ( 'NONE',  ( -39.18865352187957996, -294.0291617488275051, -195.3711623932291559 ) ) ;
#47112=CARTESIAN_POINT ( 'NONE',  ( -97.75686792767474742, -277.4148497394630795, -224.2532558495760497 ) ) ;
#47113=CARTESIAN_POINT ( 'NONE',  ( 0.9318544525416424529, -277.1785558957761282, -332.7024417860861263 ) ) ;
#47114=CARTESIAN_POINT ( 'NONE',  ( -37.28933217341737816, -285.0516177149982582, -345.5405253696986279 ) ) ;
#47116=CARTESIAN_POINT ( 'NONE',  ( -112.2421295699888759, -292.6041609144544964, -260.0152238140716463 ) ) ;
#47117=CARTESIAN_POINT ( 'NONE',  ( -102.8913616717953516, -294.0657646029418402, -306.9117459754523907 ) ) ;
#47118=CARTESIAN_POINT ( 'NONE',  ( 39.41692945656124891, -286.6926358324863031, -265.8381145829597472 ) ) ;
#47119=CARTESIAN_POINT ( 'NONE',  ( -57.85800909566775374, -290.1827263545806090, -199.4167535430180749 ) ) ;
#47121=CARTESIAN_POINT ( 'NONE',  ( -24.25815183867002389, -275.5665616661739818, -342.7320977899362902 ) ) ;
#47122=CARTESIAN_POINT ( 'NONE',  ( -10.05769737431661426, -292.8316759633332254, -339.4005898417319145 ) ) ;
#47125=CARTESIAN_POINT ( 'NONE',  ( -69.31482710721708429, -290.1189892909160335, -201.0617937484004756 ) ) ;
#47126=CARTESIAN_POINT ( 'NONE',  ( -27.75256220885212599, -287.7760919578826133, -197.1867450913030382 ) ) ;
#47127=CARTESIAN_POINT ( 'NONE',  ( -34.72446953642129586, -287.2595518301836819, -346.3027015835333486 ) ) ;
#47128=CARTESIAN_POINT ( 'NONE',  ( -88.11405299361572929, -286.7497372199761116, -217.0925240394139450 ) ) ;
#47130=CARTESIAN_POINT ( 'NONE',  ( -35.94060436001419845, -286.8730058873092048, -197.2130581441678032 ) ) ;
#47131=CARTESIAN_POINT ( 'NONE',  ( 20.92115485456609747, -294.8762410942761107, -222.5715109931754796 ) ) ;
#47132=CARTESIAN_POINT ( 'NONE',  ( -111.8826778263785400, -276.4743791852865797, -282.7286902134890738 ) ) ;
#47134=CARTESIAN_POINT ( 'NONE',  ( -89.19474017715236869, -278.0916778851050708, -327.2558148278662884 ) ) ;
#47136=CARTESIAN_POINT ( 'NONE',  ( -73.95923529058131862, -289.6494777270734176, -204.2667133945505782 ) ) ;
#47137=CARTESIAN_POINT ( 'NONE',  ( -109.7367621446333175, -278.2191181191696501, -296.7459905918261143 ) ) ;
#47138=CARTESIAN_POINT ( 'NONE',  ( -82.96900631644514590, -299.4046923507244173, -211.2194067983151342 ) ) ;
#47140=CARTESIAN_POINT ( 'NONE',  ( -112.2234160870243755, -282.6168989381570213, -265.3056901342445144 ) ) ;
#47142=CARTESIAN_POINT ( 'NONE',  ( -104.4769649845768242, -277.1141253953377941, -238.5588094975017839 ) ) ;
#47144=CARTESIAN_POINT ( 'NONE',  ( 36.17980464814537811, -279.7422620177828776, -285.1796532502651758 ) ) ;
#47146=CARTESIAN_POINT ( 'NONE',  ( -35.74559636889907921, -275.5123879625615473, -346.6640981007853384 ) ) ;
#47148=CARTESIAN_POINT ( 'NONE',  ( -107.5236829127419327, -297.7750554325476173, -293.0027641199662298 ) ) ;
#47149=CARTESIAN_POINT ( 'NONE',  ( -74.13980196493383801, -282.4493524272839409, -337.7062748260351555 ) ) ;
#47150=CARTESIAN_POINT ( 'NONE',  ( -60.60195323911070631, -298.6842837270797872, -200.8641937631643941 ) ) ;
#47151=CARTESIAN_POINT ( 'NONE',  ( -113.1156854297965992, -298.0014884745592099, -259.7020454363106978 ) ) ;
#47152=CARTESIAN_POINT ( 'NONE',  ( -40.77168706947929877, -273.6746789753167945, -197.3708606759422821 ) ) ;
#47153=CARTESIAN_POINT ( 'NONE',  ( 14.26127856995982057, -294.7774907186017117, -215.9356346469230346 ) ) ;
#47154=CARTESIAN_POINT ( 'NONE',  ( -2.224799869616333581, -286.6706045093060311, -201.8204337911280675 ) ) ;
#47155=CARTESIAN_POINT ( 'NONE',  ( 23.36354274383952401, -274.3046820923499922, -315.6951997626322850 ) ) ;
#47156=CARTESIAN_POINT ( 'NONE',  ( -9.565311140439558102, -288.5323722803806845, -342.1766610029550293 ) ) ;
#47157=CARTESIAN_POINT ( 'NONE',  ( 35.35634138105455548, -286.7273266253073416, -279.2156766240199204 ) ) ;
#47158=CARTESIAN_POINT ( 'NONE',  ( -112.2548800659922676, -288.5056641619256084, -273.9689036732924023 ) ) ;
#47160=CARTESIAN_POINT ( 'NONE',  ( -71.74250447947856912, -195.9422791308210492, -360.7315132586310824 ) ) ;
#47161=CARTESIAN_POINT ( 'NONE',  ( 22.00802344034511648, -287.6549668630858037, -312.9709613772907346 ) ) ;
#47163=CARTESIAN_POINT ( 'NONE',  ( -102.3256864906119290, -286.0301347428381860, -229.4966868831272109 ) ) ;
#47164=CARTESIAN_POINT ( 'NONE',  ( 22.03490634339488707, -291.9555696385959891, -221.7068394665944311 ) ) ;
#47165=CARTESIAN_POINT ( 'NONE',  ( -11.79693778787579816, -281.9792547514335297, -198.5150174740892339 ) ) ;
#47166=CARTESIAN_POINT ( 'NONE',  ( 30.27805885086473836, -282.4008973034112273, -234.4590241448295842 ) ) ;
#47167=CARTESIAN_POINT ( 'NONE',  ( -78.37838197559871389, -283.4550003757768764, -330.7348767477325282 ) ) ;
#47168=CARTESIAN_POINT ( 'NONE',  ( 4.264197598525720778, -278.4913503183393004, -332.7626397683217192 ) ) ;
#47169=CARTESIAN_POINT ( 'NONE',  ( -109.8508619828462400, -296.8792365744756125, -244.4493166727415030 ) ) ;
#47170=CARTESIAN_POINT ( 'NONE',  ( -34.03513793910386909, -275.4097870147164144, -196.9423865484524754 ) ) ;
#47171=CARTESIAN_POINT ( 'NONE',  ( -73.39986577598109818, -289.5918865061569818, -204.9451402227256267 ) ) ;
#47172=CARTESIAN_POINT ( 'NONE',  ( -86.29654150467598583, -296.2737638410041541, -215.7932741674931094 ) ) ;
#47175=CARTESIAN_POINT ( 'NONE',  ( -111.4301104290268825, -286.5723994601119102, -262.6242205531833633 ) ) ;
#47176=CARTESIAN_POINT ( 'NONE',  ( 27.85044064430050526, -295.1633034322525191, -310.8524654708133426 ) ) ;
#47177=CARTESIAN_POINT ( 'NONE',  ( -108.5226542122557305, -284.9836001232575313, -287.0640393276780742 ) ) ;
#47178=CARTESIAN_POINT ( 'NONE',  ( 20.63464958603786314, -275.2931151349641823, -320.6956497394458552 ) ) ;
#47179=CARTESIAN_POINT ( 'NONE',  ( -50.55700361745870453, -292.5390305648504068, -194.6071178242516169 ) ) ;
#47180=CARTESIAN_POINT ( 'NONE',  ( -111.0235649003089264, -282.4667926742456530, -288.0594715057580970 ) ) ;
#47181=CARTESIAN_POINT ( 'NONE',  ( -53.38905477198330374, -292.1851602701935917, -195.0190081488170506 ) ) ;
#47182=CARTESIAN_POINT ( 'NONE',  ( -37.26373621707863037, -289.3844316427937429, -343.3822204702021850 ) ) ;
#47185=CARTESIAN_POINT ( 'NONE',  ( -110.8432946575179585, -271.2105112503826376, -270.3440356799262645 ) ) ;
#47186=CARTESIAN_POINT ( 'NONE',  ( -113.6475361307806935, -286.0767731276364430, -270.0045470763440107 ) ) ;
#47187=CARTESIAN_POINT ( 'NONE',  ( -106.6662871844225293, -293.6237833571632336, -303.7098442033569086 ) ) ;
#47188=CARTESIAN_POINT ( 'NONE',  ( 27.12035354289720956, -280.9468365232679048, -305.2734325618674802 ) ) ;
#47189=CARTESIAN_POINT ( 'NONE',  ( 16.93730589883815085, -275.9714655962019947, -325.0206520257424359 ) ) ;
#47190=CARTESIAN_POINT ( 'NONE',  ( -105.0389662326316227, -280.9740806421274897, -238.3470921048167952 ) ) ;
#47191=CARTESIAN_POINT ( 'NONE',  ( -10.83832046195042942, -93.09808498907607088, -357.9296412820179398 ) ) ;
#47192=CARTESIAN_POINT ( 'NONE',  ( -94.90291095533092403, -282.4420381907338538, -320.6136134625443788 ) ) ;
#47193=CARTESIAN_POINT ( 'NONE',  ( -111.5099796081230181, -282.4578481200293822, -279.2292867579384961 ) ) ;
#47194=CARTESIAN_POINT ( 'NONE',  ( -9.594216685023646107, -300.1551415047837850, -194.3662611768685906 ) ) ;
#47195=CARTESIAN_POINT ( 'NONE',  ( -72.14837848031922363, -296.0180212675554117, -334.6131099744407607 ) ) ;
#47196=VERTEX_POINT ( 'NONE', #29594 ) ;
#47197=CARTESIAN_POINT ( 'NONE',  ( 2.521963754546275638, -291.2833017870509025, -208.5583619379495701 ) ) ;
#47198=CARTESIAN_POINT ( 'NONE',  ( 36.78957282834523568, -276.4605359260473847, -290.8520351895751332 ) ) ;
#47199=CARTESIAN_POINT ( 'NONE',  ( -24.59643370986773903, -274.2192078372899573, -198.4307552523208642 ) ) ;
#47200=CARTESIAN_POINT ( 'NONE',  ( 22.39154968962667880, -275.1199348831720499, -318.4800282412595038 ) ) ;
#47202=CARTESIAN_POINT ( 'NONE',  ( -89.03795467839073297, -271.3257309467421692, -215.9538867083872447 ) ) ;
#47203=CARTESIAN_POINT ( 'NONE',  ( -41.89218676549776177, -296.5335659507661035, -346.6882666136403373 ) ) ;
#47208=VECTOR ( 'NONE', #51465, 999.9999999999998863 ) ;
#47209=CARTESIAN_POINT ( 'NONE',  ( -13.41554291714954950, -283.8138374632072214, -339.7097227638931258 ) ) ;
#47210=CARTESIAN_POINT ( 'NONE',  ( 37.43248178429178097, -283.4845499658496237, -283.9537036214402406 ) ) ;
#47211=CARTESIAN_POINT ( 'NONE',  ( -107.0855911612821956, -283.6108530795273737, -292.2627693309453321 ) ) ;
#47212=CARTESIAN_POINT ( 'NONE',  ( 1.272834650735972462, -274.9273772703353416, -333.3127936274298690 ) ) ;
#47213=CARTESIAN_POINT ( 'NONE',  ( 6.337672445789625186, -284.3122010144008414, -330.3859285969235771 ) ) ;
#47214=CARTESIAN_POINT ( 'NONE',  ( -62.04026454272535318, -275.8589174673692241, -339.8465540622723893 ) ) ;
#47216=CARTESIAN_POINT ( 'NONE',  ( 20.08911706048522561, -275.9911781487510893, -224.7786915983855351 ) ) ;
#47218=VECTOR ( 'NONE', #68473, 999.9999999999998863 ) ;
#47219=CARTESIAN_POINT ( 'NONE',  ( -112.8394405884124865, -279.5349754866853687, -255.9990956565135889 ) ) ;
#47222=CARTESIAN_POINT ( 'NONE',  ( -110.6733569989350059, -286.1696982874262289, -289.4591053198163308 ) ) ;
#47223=CARTESIAN_POINT ( 'NONE',  ( -71.01419933998907652, -294.7055366935867369, -335.3271511601451493 ) ) ;
#47224=CARTESIAN_POINT ( 'NONE',  ( -112.8233061686552077, -290.0855815693317368, -255.6010678277281727 ) ) ;
#47225=CARTESIAN_POINT ( 'NONE',  ( 29.73767984930548280, -285.3754527291678755, -239.0828380946817902 ) ) ;
#47226=CARTESIAN_POINT ( 'NONE',  ( 19.98555534489466012, -285.4795617971160482, -224.2004850895096979 ) ) ;
#47227=CARTESIAN_POINT ( 'NONE',  ( -109.0852771559119674, -289.0293905106826173, -252.1208167930734589 ) ) ;
#47228=CARTESIAN_POINT ( 'NONE',  ( -108.8084297621258543, -285.5371730028592765, -287.1383326504704314 ) ) ;
#47229=CARTESIAN_POINT ( 'NONE',  ( 37.38555868714419006, -273.6340407210270200, -276.7515355555096335 ) ) ;
#47230=CARTESIAN_POINT ( 'NONE',  ( 38.84068377116534521, -285.9313171855880569, -268.7225830092211822 ) ) ;
#47231=CARTESIAN_POINT ( 'NONE',  ( 37.53100599718245434, -285.4597184642306615, -263.1588784501709029 ) ) ;
#47232=CARTESIAN_POINT ( 'NONE',  ( 27.98587816216208424, -282.0440598634750131, -237.1471077708655173 ) ) ;
#47233=CARTESIAN_POINT ( 'NONE',  ( -43.01782751543093752, -291.1238205177603504, -345.3131693545683447 ) ) ;
#47236=CARTESIAN_POINT ( 'NONE',  ( -61.11486860875385219, -297.2784201850321324, -342.1385420411614291 ) ) ;
#47237=CARTESIAN_POINT ( 'NONE',  ( -21.75454244161035433, -278.2516332032158175, -196.9454404879627418 ) ) ;
#47238=CARTESIAN_POINT ( 'NONE',  ( 26.36476417200979583, -292.1810160919434907, -227.3065301838002767 ) ) ;
#47239=CARTESIAN_POINT ( 'NONE',  ( -103.4942067497565148, -294.5120006437263100, -303.1918945326826815 ) ) ;
#47240=CARTESIAN_POINT ( 'NONE',  ( 7.456095199235232229, -279.3622530651644524, -212.0352293784813185 ) ) ;
#47241=CARTESIAN_POINT ( 'NONE',  ( 35.53605300513926579, -273.4349377660291225, -255.1281866929532782 ) ) ;
#47242=CARTESIAN_POINT ( 'NONE',  ( 32.82257019504893947, -295.1551674660261710, -292.2293288893948215 ) ) ;
#47243=CARTESIAN_POINT ( 'NONE',  ( -20.19161114001083490, -297.3376638359845288, -345.3538533559490702 ) ) ;
#47244=CARTESIAN_POINT ( 'NONE',  ( -35.47338832949255050, -296.5550266624689471, -194.0549192838901718 ) ) ;
#47245=CARTESIAN_POINT ( 'NONE',  ( -33.50867054411274637, -293.2444201040388521, -346.2639976651822167 ) ) ;
#47246=CARTESIAN_POINT ( 'NONE',  ( 17.16247376825644366, -294.2739021256037972, -220.8427991493268507 ) ) ;
#47249=CARTESIAN_POINT ( 'NONE',  ( 24.98007436116651903, -293.8267322415183003, -231.9426701240216744 ) ) ;
#47250=CARTESIAN_POINT ( 'NONE',  ( -6.159652433930307147, -280.6645610799988049, -338.9620415035131487 ) ) ;
#47251=CARTESIAN_POINT ( 'NONE',  ( -67.29520944067623134, -295.4562114322068851, -336.9464943259771985 ) ) ;
#47252=CARTESIAN_POINT ( 'NONE',  ( -37.31425204684190078, -283.0517811524608760, -347.3741783324445578 ) ) ;
#47253=CARTESIAN_POINT ( 'NONE',  ( -114.3053226495254080, -284.2595292315277220, -267.1110651571665358 ) ) ;
#47254=CARTESIAN_POINT ( 'NONE',  ( -93.81153541482309777, -287.8683913136264323, -319.5424193463255733 ) ) ;
#47257=CARTESIAN_POINT ( 'NONE',  ( -19.10304683103889545, -281.3015717310748869, -344.5105118003510825 ) ) ;
#47258=CARTESIAN_POINT ( 'NONE',  ( -8.362728976432034500, -287.6018775804433290, -341.3803378083374582 ) ) ;
#47260=CARTESIAN_POINT ( 'NONE',  ( -84.97912683419076529, -297.3220132842349699, -326.7941103515584018 ) ) ;
#47261=CARTESIAN_POINT ( 'NONE',  ( -14.74647924161341983, -278.1903711024790482, -343.4100976707210862 ) ) ;
#47262=CARTESIAN_POINT ( 'NONE',  ( -6.756690381603299045, -280.1317573073408198, -204.0402689355569521 ) ) ;
#47263=CARTESIAN_POINT ( 'NONE',  ( -34.96253972944582245, -292.2479057605982575, -193.3847325202386571 ) ) ;
#47264=CARTESIAN_POINT ( 'NONE',  ( -16.56177522502391142, -280.8656932031627207, -343.0618293177664100 ) ) ;
#47265=CARTESIAN_POINT ( 'NONE',  ( -9.627357516935083126, -291.4819615835115769, -202.5183384911460109 ) ) ;
#47266=CARTESIAN_POINT ( 'NONE',  ( -112.3662713181513766, -294.5259416601297175, -272.3896070059856243 ) ) ;
#47270=CARTESIAN_POINT ( 'NONE',  ( 21.37218548273926189, -293.6689582017637008, -313.8429311725598723 ) ) ;
#47272=CARTESIAN_POINT ( 'NONE',  ( -37.37352853689063181, -292.5523547857346784, -340.3611179825599606 ) ) ;
#47273=CARTESIAN_POINT ( 'NONE',  ( -110.8795906677379151, -272.0316282877120102, -247.9006872612312691 ) ) ;
#47274=CARTESIAN_POINT ( 'NONE',  ( 36.13918005954949564, -279.4569759122437063, -251.8985685792554250 ) ) ;
#47275=CARTESIAN_POINT ( 'NONE',  ( -68.31654884858404841, -286.9689080755973691, -200.3907242899047105 ) ) ;
#47276=CARTESIAN_POINT ( 'NONE',  ( -8.220444392594361105, -288.4933151116125600, -337.3550734263518507 ) ) ;
#47277=CARTESIAN_POINT ( 'NONE',  ( -110.8516076071489209, -280.1401837666065830, -265.1648449456408798 ) ) ;
#47278=CARTESIAN_POINT ( 'NONE',  ( -37.16945262842013875, -299.8144870652361078, -196.3448372581566730 ) ) ;
#47279=CARTESIAN_POINT ( 'NONE',  ( -89.37810487790241609, -276.5996840815217297, -322.1956765249523187 ) ) ;
#47281=CARTESIAN_POINT ( 'NONE',  ( -114.3416212705230350, -272.4213605645363145, -267.4915351304622391 ) ) ;
#47282=CARTESIAN_POINT ( 'NONE',  ( -101.5335610857579240, -291.9635430976080670, -308.1550172619818682 ) ) ;
#47283=CARTESIAN_POINT ( 'NONE',  ( 21.57758991090565814, -294.4965387587181453, -222.0397181733385992 ) ) ;
#47285=CARTESIAN_POINT ( 'NONE',  ( -109.7227076263855849, -291.0674761955495455, -280.6920631529058028 ) ) ;
#47287=CARTESIAN_POINT ( 'NONE',  ( 33.31955561591752257, -291.3381369091403030, -242.8793666042133168 ) ) ;
#47288=CARTESIAN_POINT ( 'NONE',  ( -57.38830422467615477, -298.1337010959110216, -195.9830581277876433 ) ) ;
#47291=CARTESIAN_POINT ( 'NONE',  ( -107.7350601565815538, -292.4502854101468188, -240.9080601619868105 ) ) ;
#47292=CARTESIAN_POINT ( 'NONE',  ( -72.08107566293803359, -294.1233781216987495, -198.2974183793908196 ) ) ;
#47294=CARTESIAN_POINT ( 'NONE',  ( -111.6912696969639995, -286.4372592251715446, -279.3020659056818999 ) ) ;
#47295=CARTESIAN_POINT ( 'NONE',  ( 8.472924297440355801, -272.6810440886767424, -211.1914584251230735 ) ) ;
#47296=CARTESIAN_POINT ( 'NONE',  ( -18.93882080572176108, -276.2109099559589822, -198.1782757031507174 ) ) ;
#47297=CARTESIAN_POINT ( 'NONE',  ( -5.402030447738578545, -290.5555130453395805, -203.1074028878531976 ) ) ;
#47298=CARTESIAN_POINT ( 'NONE',  ( -96.94232405863537849, -279.7770074085086662, -317.1379403594822293 ) ) ;
#47301=CARTESIAN_POINT ( 'NONE',  ( -46.45645791131997271, -279.9334011040078849, -197.8812840090843963 ) ) ;
#47302=CARTESIAN_POINT ( 'NONE',  ( 31.44770197111118648, -281.2314993360548669, -295.2475694520865090 ) ) ;
#47303=CARTESIAN_POINT ( 'NONE',  ( -25.80285307207096679, -277.9881240492748589, -346.1789754943714001 ) ) ;
#47304=CARTESIAN_POINT ( 'NONE',  ( 39.13170861255787258, -280.4135515326923951, -275.6488589930308990 ) ) ;
#47305=CARTESIAN_POINT ( 'NONE',  ( 183.2382489426448444, 261.9115828407970525, -151.4279635117714804 ) ) ;
#47306=CARTESIAN_POINT ( 'NONE',  ( 4.724172336070187939, -275.5461014643733506, -206.0852640459838767 ) ) ;
#47308=CARTESIAN_POINT ( 'NONE',  ( -46.81429039673593451, -275.4540674548663901, -194.6446878945457968 ) ) ;
#47309=CARTESIAN_POINT ( 'NONE',  ( -92.05005921254146983, -280.4090924074130839, -314.0302885647153062 ) ) ;
#47312=CARTESIAN_POINT ( 'NONE',  ( -23.71428578425187084, -289.9537248085028409, -342.4444172017016399 ) ) ;
#47313=CARTESIAN_POINT ( 'NONE',  ( 37.11984029285012809, -289.5042570858722115, -285.5088245613155209 ) ) ;
#47314=CARTESIAN_POINT ( 'NONE',  ( -73.60272487931625562, -288.8955944053112148, -333.8501968845516217 ) ) ;
#47315=CARTESIAN_POINT ( 'NONE',  ( -10.00995263068972996, -285.9071430336842354, -198.3842487652408977 ) ) ;
#47317=CARTESIAN_POINT ( 'NONE',  ( 18.19357468365641495, -280.6380219744269766, -318.9643449126352834 ) ) ;
#47318=CARTESIAN_POINT ( 'NONE',  ( 23.78014919883603895, -289.9897879115958403, -312.5141052227509135 ) ) ;
#47319=CARTESIAN_POINT ( 'NONE',  ( -78.78235003413496429, -282.1017764170376836, -331.2986293077425444 ) ) ;
#47320=CARTESIAN_POINT ( 'NONE',  ( -109.6201222492224758, -280.0416918402560214, -257.0542334995348597 ) ) ;
#47321=CARTESIAN_POINT ( 'NONE',  ( -48.61115109039207738, -277.6917294630731590, -342.5997224945263042 ) ) ;
#47323=CARTESIAN_POINT ( 'NONE',  ( -102.8681893677457424, -289.8687932627612440, -230.5815831281811086 ) ) ;
#47324=CARTESIAN_POINT ( 'NONE',  ( -69.73410099337527868, -286.4392955085043013, -200.6697328347086113 ) ) ;
#47325=CARTESIAN_POINT ( 'NONE',  ( -37.98822370681094185, -286.5365997589728977, -193.4253726438971626 ) ) ;
#47326=CARTESIAN_POINT ( 'NONE',  ( -110.3093882375007553, -284.7474822887779169, -268.1893683537275592 ) ) ;
#47329=CARTESIAN_POINT ( 'NONE',  ( -94.51045356221453630, -291.7295095897889610, -320.0807229001769656 ) ) ;
#47331=CARTESIAN_POINT ( 'NONE',  ( 30.45753330345767296, -292.6972775638323583, -305.8091393317166080 ) ) ;
#47332=CARTESIAN_POINT ( 'NONE',  ( -2.792100925336592265, -273.5795401780071643, -205.7876432151709309 ) ) ;
#47333=CARTESIAN_POINT ( 'NONE',  ( -58.83080049629687380, -294.6714826667498528, -344.2511044763451196 ) ) ;
#47334=CARTESIAN_POINT ( 'NONE',  ( -65.57485277101740451, -290.1560276251775576, -202.2769488683008774 ) ) ;
#47335=CARTESIAN_POINT ( 'NONE',  ( -39.74407791727685435, -293.3225587706272677, -344.3480581158621590 ) ) ;
#47337=CARTESIAN_POINT ( 'NONE',  ( -80.62938103434809989, -290.8587372268113427, -329.6975100401652981 ) ) ;
#47338=CARTESIAN_POINT ( 'NONE',  ( 128.9467878515196162, -299.5541904835127980, -195.3611179825600175 ) ) ;
#47340=CARTESIAN_POINT ( 'NONE',  ( 9.984731590192005513, -290.7018841867899823, -211.8968966108954248 ) ) ;
#47341=CARTESIAN_POINT ( 'NONE',  ( -31.29466985583038863, -296.9760661300392144, -345.1681882278454623 ) ) ;
#47342=CARTESIAN_POINT ( 'NONE',  ( 26.56687212397964259, -288.0045184762986423, -234.4928423007621063 ) ) ;
#47343=CONICAL_SURFACE ( 'NONE', #66982, 6.249455242036738412, 0.09862129276975223346 ) ;
#47344=CARTESIAN_POINT ( 'NONE',  ( 24.77415395929567055, -276.9564266500975691, -227.6764777438025931 ) ) ;
#47345=CARTESIAN_POINT ( 'NONE',  ( -31.49596081180238016, -275.7749559887330406, -346.7930225799743766 ) ) ;
#47346=CARTESIAN_POINT ( 'NONE',  ( -65.47334378413312095, -296.8908782242624511, -198.8006192232170122 ) ) ;
#47347=CARTESIAN_POINT ( 'NONE',  ( 36.61327719983081863, -273.8444212658760648, -274.3898287576024586 ) ) ;
#47348=CARTESIAN_POINT ( 'NONE',  ( -93.27458176858496586, -277.3197769015390008, -221.2212000298078465 ) ) ;
#47349=CARTESIAN_POINT ( 'NONE',  ( -90.49468936121647289, -274.4833408100532779, -219.7276072861770615 ) ) ;
#47350=CARTESIAN_POINT ( 'NONE',  ( -9.523053172182095238, -275.0944882167575543, -341.3016797020646322 ) ) ;
#47354=CARTESIAN_POINT ( 'NONE',  ( -67.10659532917318870, -274.3027702877292882, -203.5795708894461882 ) ) ;
#47356=CARTESIAN_POINT ( 'NONE',  ( -12.78409989859064666, -286.7547538235076559, -341.6571463136292550 ) ) ;
#47357=CARTESIAN_POINT ( 'NONE',  ( 32.86060664846892365, -275.1186717630363319, -250.1645787173510485 ) ) ;
#47359=CARTESIAN_POINT ( 'NONE',  ( 35.07247007989381160, -287.8844780226338003, -296.6923417897996842 ) ) ;
#47360=CARTESIAN_POINT ( 'NONE',  ( -80.53226247933328352, -289.2866503103895184, -334.1461522656327361 ) ) ;
#47361=CARTESIAN_POINT ( 'NONE',  ( 28.95563896395952597, -300.8580694568498757, -194.9836664655143181 ) ) ;
#47362=CARTESIAN_POINT ( 'NONE',  ( -101.4546696032397364, -295.0712285559720840, -231.6656413759651798 ) ) ;
#47363=CARTESIAN_POINT ( 'NONE',  ( 37.03293015940866439, -280.9914175798062956, -289.6632730590859524 ) ) ;
#47365=CARTESIAN_POINT ( 'NONE',  ( -106.9091457518933197, -276.1851947626889228, -298.5227303991360372 ) ) ;
#47368=CARTESIAN_POINT ( 'NONE',  ( -107.3353889128277245, -289.0538256479035226, -292.6203719295008341 ) ) ;
#47371=CARTESIAN_POINT ( 'NONE',  ( -111.6790434902572571, -288.6846530815898859, -260.0290238052101586 ) ) ;
#47372=CARTESIAN_POINT ( 'NONE',  ( -19.11871989594659738, -275.8109422362250029, -198.9034994426666287 ) ) ;
#47373=CARTESIAN_POINT ( 'NONE',  ( 39.05077414529836943, -282.9358772276694367, -267.0645545634561699 ) ) ;
#47374=CARTESIAN_POINT ( 'NONE',  ( -33.41547829631709732, -296.1211820599642124, -195.0072265337391002 ) ) ;
#47375=CARTESIAN_POINT ( 'NONE',  ( -86.92883687992903674, -283.7652306175546073, -324.0037369043731132 ) ) ;
#47376=CARTESIAN_POINT ( 'NONE',  ( -59.67157749833192071, -275.1826000562756462, -200.1882128524400741 ) ) ;
#47377=CARTESIAN_POINT ( 'NONE',  ( 23.92314449272920740, -275.8020554696799422, -230.3708624129477585 ) ) ;
#47378=CARTESIAN_POINT ( 'NONE',  ( 20.37299723747537428, -286.3015841687665670, -319.1292213796348847 ) ) ;
#47380=CARTESIAN_POINT ( 'NONE',  ( -30.37464905788779390, -284.9641743501232440, -345.0368225177737713 ) ) ;
#47381=CARTESIAN_POINT ( 'NONE',  ( -109.4311415970967829, -271.6509713783288475, -256.7729986090099601 ) ) ;
#47383=CARTESIAN_POINT ( 'NONE',  ( 204.9610684336733186, 293.7029684379119772, -54.00000000001035971 ) ) ;
#47384=CARTESIAN_POINT ( 'NONE',  ( 39.60680653321302458, -293.4206848386472188, -273.1766689201677423 ) ) ;
#47385=CARTESIAN_POINT ( 'NONE',  ( -107.1110617080529863, -286.8785060076702393, -243.8265558891319529 ) ) ;
#47389=CARTESIAN_POINT ( 'NONE',  ( -111.2586520408596868, -270.4809262143062369, -234.7283546768995564 ) ) ;
#47390=CARTESIAN_POINT ( 'NONE',  ( -103.4720422245554801, -277.2373635576383890, -309.5926677842815593 ) ) ;
#47391=CARTESIAN_POINT ( 'NONE',  ( -112.0873016528295523, -288.7639433271329494, -285.2440726262187809 ) ) ;
#47392=CARTESIAN_POINT ( 'NONE',  ( -21.21783944934228217, -284.3618259955413237, -342.3214079021063867 ) ) ;
#47393=CARTESIAN_POINT ( 'NONE',  ( -100.0214892336160233, -279.7750505408614003, -309.8169143988872065 ) ) ;
#47394=CARTESIAN_POINT ( 'NONE',  ( -103.5391334409621464, -286.4785562596400723, -232.0916561192736935 ) ) ;
#47395=CARTESIAN_POINT ( 'NONE',  ( -3.466408484041502813, -282.4994331433874777, -203.4329837190015269 ) ) ;
#47396=CARTESIAN_POINT ( 'NONE',  ( -0.04730437892725614796, -274.7009416561237458, -202.9804953923291464 ) ) ;
#47397=CARTESIAN_POINT ( 'NONE',  ( -113.7665136220991116, -278.2627065904239885, -280.1773941270806176 ) ) ;
#47399=CARTESIAN_POINT ( 'NONE',  ( -80.97954547535800884, -297.5700992779682679, -330.6690996157812492 ) ) ;
#47402=CARTESIAN_POINT ( 'NONE',  ( -20.82146376237103880, -296.3964595977623162, -194.6014795725925524 ) ) ;
#47403=CARTESIAN_POINT ( 'NONE',  ( 29.14464829593334017, -274.6502850783444956, -239.9475571715804563 ) ) ;
#47405=CARTESIAN_POINT ( 'NONE',  ( 7.749300273335740563, -299.6839338148757292, -193.6621707208877012 ) ) ;
#47406=CARTESIAN_POINT ( 'NONE',  ( -42.77051783036284860, -287.7428939757972444, -196.5343485453171297 ) ) ;
#47407=CARTESIAN_POINT ( 'NONE',  ( -55.88291227595162525, -296.8068188998313417, -344.3809207585816239 ) ) ;
#47408=CARTESIAN_POINT ( 'NONE',  ( -109.0603444146798324, -297.4132932125892808, -297.4262036220541745 ) ) ;
#47409=CARTESIAN_POINT ( 'NONE',  ( -110.5083084155153443, -292.7544217070788477, -254.6551999153137160 ) ) ;
#47410=CARTESIAN_POINT ( 'NONE',  ( 3.730982949472132493, -278.6056800005169407, -207.7444452180383792 ) ) ;
#47411=CIRCLE ( 'NONE', #88249, 2.397123461337413719 ) ;
#47412=CARTESIAN_POINT ( 'NONE',  ( -99.20366507609693940, -281.0373173936168314, -228.8640943438021793 ) ) ;
#47413=CARTESIAN_POINT ( 'NONE',  ( -35.75314610685270367, -296.1520347558109734, -195.9216345540877739 ) ) ;
#47414=CARTESIAN_POINT ( 'NONE',  ( -66.08534010418512139, -285.2847250274622297, -340.4757777030929446 ) ) ;
#47415=CARTESIAN_POINT ( 'NONE',  ( 31.68585556289645666, -286.7997918608118653, -295.0476047435032569 ) ) ;
#47416=CARTESIAN_POINT ( 'NONE',  ( 26.96909223665486621, -23.88996772622144249, -344.7745201028783413 ) ) ;
#47418=CARTESIAN_POINT ( 'NONE',  ( -38.62102233416989350, -285.7024252220199401, -197.3386961749848183 ) ) ;
#47420=CARTESIAN_POINT ( 'NONE',  ( -35.89119930362267752, -284.1140596053600120, -347.0513531479867311 ) ) ;
#47421=CARTESIAN_POINT ( 'NONE',  ( -106.3277506709990092, -273.2036926250512465, -246.4234422967631986 ) ) ;
#47422=CARTESIAN_POINT ( 'NONE',  ( -18.26599194427078032, -285.0874671611159101, -196.1164992782853176 ) ) ;
#47423=CARTESIAN_POINT ( 'NONE',  ( -17.06571014245249529, -281.2489917871808416, -196.3225844852802311 ) ) ;
#47425=CARTESIAN_POINT ( 'NONE',  ( -110.6763272792857435, -280.3390741257584295, -249.2722532903270292 ) ) ;
#47426=CARTESIAN_POINT ( 'NONE',  ( 3.807081742047634609, -280.9228225300652184, -205.2403197321870607 ) ) ;
#47427=CARTESIAN_POINT ( 'NONE',  ( -53.28691492658257545, -289.3380690714490129, -200.3538533559491555 ) ) ;
#47428=CARTESIAN_POINT ( 'NONE',  ( -99.18224766838898177, -248.6449173048312105, -334.3546491526849991 ) ) ;
#47430=CARTESIAN_POINT ( 'NONE',  ( -29.83056001419215519, -276.1476309348029758, -195.9056870182791386 ) ) ;
#47431=CARTESIAN_POINT ( 'NONE',  ( -13.44854438592516743, -91.33897161315739766, -359.8347524150512413 ) ) ;
#47433=CARTESIAN_POINT ( 'NONE',  ( 33.79121296540559882, -279.8676103630207308, -293.1557082655626800 ) ) ;
#47434=CARTESIAN_POINT ( 'NONE',  ( -27.99624598022954913, -293.9292366935629843, -194.8983609080697192 ) ) ;
#47435=CARTESIAN_POINT ( 'NONE',  ( -37.00339734540678904, -294.3963586086436521, -343.4747099381384601 ) ) ;
#47436=CARTESIAN_POINT ( 'NONE',  ( -107.2019207893588231, -290.4739283764644142, -237.9994977240889114 ) ) ;
#47437=CARTESIAN_POINT ( 'NONE',  ( -107.1748277085148118, -264.8307257489140625, -305.4825756969800068 ) ) ;
#47438=CARTESIAN_POINT ( 'NONE',  ( -112.5558899282725491, -295.2966404529260558, -256.8914503373235334 ) ) ;
#47439=CARTESIAN_POINT ( 'NONE',  ( 33.07081732972576305, -286.2437860648411743, -292.6334883398951661 ) ) ;
#47440=CARTESIAN_POINT ( 'NONE',  ( 13.21311059842174451, -296.1972275886332682, -324.7922102373204893 ) ) ;
#47441=CARTESIAN_POINT ( 'NONE',  ( 33.50911789645265770, -285.9806498269613257, -250.8315234100532791 ) ) ;
#47442=CARTESIAN_POINT ( 'NONE',  ( -109.9831983042996058, -285.7168804234313484, -281.8431347602841583 ) ) ;
#47444=CARTESIAN_POINT ( 'NONE',  ( 39.42026268742862527, -294.4566775741820948, -267.4335819055772276 ) ) ;
#47445=CARTESIAN_POINT ( 'NONE',  ( -6.000861196347877069, -283.1211577672743829, -336.3729125533952811 ) ) ;
#47446=CARTESIAN_POINT ( 'NONE',  ( -64.14171714688964698, -294.1890833164350738, -342.1230006651120448 ) ) ;
#47447=AXIS2_PLACEMENT_3D ( 'NONE', #12245, #83739, #61065 ) ;
#47448=CARTESIAN_POINT ( 'NONE',  ( -112.4054015943029583, -291.1492005077801082, -286.7806046825298267 ) ) ;
#47449=CARTESIAN_POINT ( 'NONE',  ( -56.17979313988788448, -292.3082557503146859, -195.7096097580475771 ) ) ;
#47450=CARTESIAN_POINT ( 'NONE',  ( -105.1122525118403104, -290.3540714552113400, -297.6289009731979718 ) ) ;
#47453=CARTESIAN_POINT ( 'NONE',  ( -107.2263898719252069, -298.0327134352918392, -299.7617222634390828 ) ) ;
#47454=CARTESIAN_POINT ( 'NONE',  ( -24.21248841555564013, -273.0110100372268107, -194.8378147414888133 ) ) ;
#47456=CARTESIAN_POINT ( 'NONE',  ( -68.61291896196424034, -278.6894964789363485, -204.1378643508918458 ) ) ;
#47458=CARTESIAN_POINT ( 'NONE',  ( 39.49327698980793144, -274.9983360849891483, -265.4499592058275539 ) ) ;
#47459=CARTESIAN_POINT ( 'NONE',  ( -108.1199337881546398, -295.3009131489678225, -249.8391932867297385 ) ) ;
#47460=CARTESIAN_POINT ( 'NONE',  ( -87.92008665302070369, -279.6289079625661884, -324.6997993695976561 ) ) ;
#47461=CARTESIAN_POINT ( 'NONE',  ( -11.03063068004470004, -272.5382379393943211, -200.8900630760448962 ) ) ;
#47462=CARTESIAN_POINT ( 'NONE',  ( -5.354663166924825468, -295.8266930832711523, -336.4352807222431352 ) ) ;
#47463=CARTESIAN_POINT ( 'NONE',  ( -101.4916713185849488, -298.1147185321518123, -234.8786255520706732 ) ) ;
#47465=CARTESIAN_POINT ( 'NONE',  ( -75.39822371242237864, -299.1540508785749353, -204.2843317397194198 ) ) ;
#47466=CARTESIAN_POINT ( 'NONE',  ( -29.27895349601016406, -296.1527012719359391, -195.1971838205473375 ) ) ;
#47467=CARTESIAN_POINT ( 'NONE',  ( 26.31924943952492768, -293.7111588374173721, -234.3248415415681336 ) ) ;
#47468=CARTESIAN_POINT ( 'NONE',  ( -105.2397746907739986, -289.5060556926109712, -241.8520794767093776 ) ) ;
#47469=CARTESIAN_POINT ( 'NONE',  ( 6.501289990623595472, -300.6011461931510667, -195.3461625447490917 ) ) ;
#47470=CARTESIAN_POINT ( 'NONE',  ( 4.824189293165201953, -275.0972689818939330, -205.9429204830475157 ) ) ;
#47471=CARTESIAN_POINT ( 'NONE',  ( -93.77973342082707120, -273.3749006517828661, -224.0409410538604504 ) ) ;
#47472=CARTESIAN_POINT ( 'NONE',  ( -2.374504463421271083, -284.5716752170822588, -337.1121631646437891 ) ) ;
#47473=CARTESIAN_POINT ( 'NONE',  ( -66.40452724787992622, -282.1096478607734639, -341.1470334836013762 ) ) ;
#47474=CARTESIAN_POINT ( 'NONE',  ( -45.64686461744222612, -276.5032441622067836, -346.8623701648375004 ) ) ;
#47476=CARTESIAN_POINT ( 'NONE',  ( -108.2522530744371210, -283.5121569656338920, -288.3693163455671424 ) ) ;
#47477=CARTESIAN_POINT ( 'NONE',  ( 35.89710774520484193, -279.3346401882822647, -253.3898294352219125 ) ) ;
#47479=CARTESIAN_POINT ( 'NONE',  ( 36.18973025653325948, -274.1792362902468199, -274.3626201796190571 ) ) ;
#47480=CARTESIAN_POINT ( 'NONE',  ( -21.29540734494232268, -278.8466385558581919, -343.6769882151688194 ) ) ;
#47483=CARTESIAN_POINT ( 'NONE',  ( -111.6584955308033216, -271.1648000688354614, -253.5250157027853959 ) ) ;
#47485=CARTESIAN_POINT ( 'NONE',  ( -61.78514788984986694, -279.3691083284649608, -341.4973439075864121 ) ) ;
#47487=CARTESIAN_POINT ( 'NONE',  ( -66.00687912452282546, -285.3444535061283318, -340.2865640699754408 ) ) ;
#47491=CARTESIAN_POINT ( 'NONE',  ( 35.60531716339978203, -285.7764613812878451, -287.8429838378509658 ) ) ;
#47493=CARTESIAN_POINT ( 'NONE',  ( -110.6389998346100185, -295.2968748261232008, -274.1868675226101573 ) ) ;
#47494=CARTESIAN_POINT ( 'NONE',  ( 4.288016781803740685, -286.6242855029354928, -331.8871624122991193 ) ) ;
#47495=CARTESIAN_POINT ( 'NONE',  ( 197.0349383350915105, 285.8449894349855640, -111.9383547020201064 ) ) ;
#47496=CARTESIAN_POINT ( 'NONE',  ( -109.3733055791940956, -294.8209521514482958, -249.4697689045983680 ) ) ;
#47497=CARTESIAN_POINT ( 'NONE',  ( -18.33583071450935620, -284.7724716257929458, -196.4046497857824818 ) ) ;
#47498=CARTESIAN_POINT ( 'NONE',  ( 20.28809305134553753, -282.5080102124807127, -224.2607128227005830 ) ) ;
#47499=CARTESIAN_POINT ( 'NONE',  ( -95.50927080877582398, -282.1247238825616819, -319.2740768333006827 ) ) ;
#47500=CARTESIAN_POINT ( 'NONE',  ( -104.0477169485465652, -290.1514632624219416, -300.1390707392179138 ) ) ;
#47503=CARTESIAN_POINT ( 'NONE',  ( -103.9105531645786584, -280.3992849684564135, -238.8731022798182835 ) ) ;
#47504=CARTESIAN_POINT ( 'NONE',  ( 2.784022759097974919, -281.4082215602958286, -209.1241289755912760 ) ) ;
#47505=EDGE_CURVE ( 'NONE', #81416, #25769, #11842, .T. ) ;
#47506=CARTESIAN_POINT ( 'NONE',  ( 36.66986701849825181, -289.3510003499635559, -256.1944410992196595 ) ) ;
#47508=CARTESIAN_POINT ( 'NONE',  ( -105.6089422716172948, -273.0129119305963172, -234.6286964650097957 ) ) ;
#47509=CARTESIAN_POINT ( 'NONE',  ( -95.58990173591513440, -293.1773796353858188, -223.6611051430612065 ) ) ;
#47511=CARTESIAN_POINT ( 'NONE',  ( -115.3288506153726871, -292.8376638359844719, -288.1938231032136741 ) ) ;
#47513=CARTESIAN_POINT ( 'NONE',  ( -28.83444490674152760, -274.9445047091547849, -345.0971162895368707 ) ) ;
#47515=CARTESIAN_POINT ( 'NONE',  ( -16.74293211478747878, -293.1904063318108911, -343.7787817393394221 ) ) ;
#47516=CARTESIAN_POINT ( 'NONE',  ( -75.23720573856124361, -297.0402515931730818, -207.8371213331801073 ) ) ;
#47517=CARTESIAN_POINT ( 'NONE',  ( -82.96044504382304297, -291.2096642047586101, -328.2371740230512387 ) ) ;
#47519=CARTESIAN_POINT ( 'NONE',  ( -68.18651957364731686, -285.2230515667905024, -337.6409153176431346 ) ) ;
#47520=CARTESIAN_POINT ( 'NONE',  ( -79.28625121524561337, -292.9236369733330321, -206.4287680954979578 ) ) ;
#47521=CARTESIAN_POINT ( 'NONE',  ( -50.49812231399131690, -293.2026845073552295, -194.9939711158508544 ) ) ;
#47522=CARTESIAN_POINT ( 'NONE',  ( -65.32499675398028671, -291.5092509534115948, -202.9240539062371056 ) ) ;
#47523=CARTESIAN_POINT ( 'NONE',  ( -27.60135774694489541, -288.1760595989682656, -195.9962984954004810 ) ) ;
#47524=CARTESIAN_POINT ( 'NONE',  ( 15.15978232629504241, -280.9352679105275570, -213.9624445336816336 ) ) ;
#47525=CARTESIAN_POINT ( 'NONE',  ( -104.6855990875592397, -294.1810387019559130, -304.7417875851074314 ) ) ;
#47526=CARTESIAN_POINT ( 'NONE',  ( -0.3773029460514870648, -282.4080053068450979, -337.9233243674437972 ) ) ;
#47527=CARTESIAN_POINT ( 'NONE',  ( 27.70765615082352440, -276.9308217806917014, -234.4846887558680351 ) ) ;
#47529=CARTESIAN_POINT ( 'NONE',  ( -105.5937364680635966, -281.2662352645559167, -254.8156830097664738 ) ) ;
#47530=CARTESIAN_POINT ( 'NONE',  ( -99.46647925246774946, -276.1091365146644421, -313.7295085455024832 ) ) ;
#47532=CARTESIAN_POINT ( 'NONE',  ( -8.475693163766912619, -282.1714385259087408, -337.4784934059893544 ) ) ;
#47533=CARTESIAN_POINT ( 'NONE',  ( -25.47232795450291221, -281.4052851904296517, -194.6833357616488343 ) ) ;
#47534=CARTESIAN_POINT ( 'NONE',  ( -89.71692275410507023, -284.3938785119666477, -214.1670333773750770 ) ) ;
#47535=CARTESIAN_POINT ( 'NONE',  ( -6.873294218886489837, -294.2177812038362958, -202.9100226822693571 ) ) ;
#47536=CARTESIAN_POINT ( 'NONE',  ( 26.25157757958301374, -276.5944132812682597, -228.3809387848266397 ) ) ;
#47537=CARTESIAN_POINT ( 'NONE',  ( 11.45817441120040314, -276.0274606959614516, -211.3697081764578911 ) ) ;
#47538=CARTESIAN_POINT ( 'NONE',  ( 7.578722814606958735, -276.2531303639588032, -327.9681698734675024 ) ) ;
#47539=CARTESIAN_POINT ( 'NONE',  ( -85.64246906516477509, -297.7219809988185375, -327.5873719487264566 ) ) ;
#47540=CARTESIAN_POINT ( 'NONE',  ( -73.23143963290321778, -283.5750233033973586, -204.6810684702057017 ) ) ;
#47541=CARTESIAN_POINT ( 'NONE',  ( 36.68499868472477488, -292.9535894915959489, -249.1992875222266832 ) ) ;
#47542=CARTESIAN_POINT ( 'NONE',  ( 37.32847133688010643, -289.3442701305405649, -285.5534157374442543 ) ) ;
#47543=CARTESIAN_POINT ( 'NONE',  ( 21.24910357455268795, -291.8563801456648434, -226.3004348748939094 ) ) ;
#47544=ORIENTED_EDGE ( 'NONE', *, *, #78765, .T. ) ;
#47545=CARTESIAN_POINT ( 'NONE',  ( 1.416997135172548106, -291.1337252148142625, -204.4495259250804509 ) ) ;
#47546=CARTESIAN_POINT ( 'NONE',  ( 26.25505679491628186, -292.7266229670518101, -234.3755570041977876 ) ) ;
#47548=CARTESIAN_POINT ( 'NONE',  ( -57.19755612380235732, -290.3820500497033663, -344.4918889757568081 ) ) ;
#47549=CARTESIAN_POINT ( 'NONE',  ( -108.6283233598747699, -279.0947672837481264, -254.4828375281031470 ) ) ;
#47550=CARTESIAN_POINT ( 'NONE',  ( -109.1529620085846943, -295.1289140791500358, -297.4300669584623051 ) ) ;
#47551=CARTESIAN_POINT ( 'NONE',  ( -71.02906988141430134, -286.2706121519483986, -201.2346114436066387 ) ) ;
#47552=CARTESIAN_POINT ( 'NONE',  ( -29.46932064590940215, -286.4825686396810625, -193.7858613210267151 ) ) ;
#47553=CARTESIAN_POINT ( 'NONE',  ( -99.04663183502438528, -284.3448762203460092, -309.5017538438171982 ) ) ;
#47554=CARTESIAN_POINT ( 'NONE',  ( 203.1405228849236551, 295.9636489450776367, -54.00000000004142464 ) ) ;
#47555=CARTESIAN_POINT ( 'NONE',  ( -91.06148389132593479, -229.3667599500281256, -346.6633138930380937 ) ) ;
#47556=CARTESIAN_POINT ( 'NONE',  ( 178.6937129019192412, 251.6256410920926214, -164.2356949225344067 ) ) ;
#47557=CARTESIAN_POINT ( 'NONE',  ( 32.21852534477521601, -274.4472130652386568, -247.5270200052369489 ) ) ;
#47558=CARTESIAN_POINT ( 'NONE',  ( 25.63411541957023587, -274.9862526052712610, -307.8880780139328408 ) ) ;
#47559=CARTESIAN_POINT ( 'NONE',  ( -113.5399384530185500, -296.1942588607597600, -259.6190226704199517 ) ) ;
#47560=CARTESIAN_POINT ( 'NONE',  ( 85.70268185674719064, 81.17150233424827377, -299.2961519048424179 ) ) ;
#47561=CARTESIAN_POINT ( 'NONE',  ( 0.7866359285302773063, -275.2399191282585207, -336.7501424353915809 ) ) ;
#47562=CARTESIAN_POINT ( 'NONE',  ( -108.1727679605407815, -274.5947437918048308, -248.7160093815739117 ) ) ;
#47564=CARTESIAN_POINT ( 'NONE',  ( -87.84319746015545149, -274.4455869132079329, -212.5748954210873478 ) ) ;
#47565=CARTESIAN_POINT ( 'NONE',  ( -108.7720538813131697, -291.2468524401055561, -255.0088215890920935 ) ) ;
#47566=CARTESIAN_POINT ( 'NONE',  ( -90.59278332608258211, -296.5861977347719858, -325.8282333287130541 ) ) ;
#47567=CARTESIAN_POINT ( 'NONE',  ( -112.8295280142959598, -297.2314629928028467, -255.4234104085188903 ) ) ;
#47568=CARTESIAN_POINT ( 'NONE',  ( -42.38760562295917111, -295.2842404874551789, -343.1865176879359751 ) ) ;
#47570=VECTOR ( 'NONE', #65848, 1000.000000000000000 ) ;
#47571=CARTESIAN_POINT ( 'NONE',  ( -25.96224266893775479, -278.8284713593610604, -345.0593250816299360 ) ) ;
#47573=CARTESIAN_POINT ( 'NONE',  ( -45.26079598530847647, -279.4621824805769847, -193.7783404584913001 ) ) ;
#47574=CARTESIAN_POINT ( 'NONE',  ( 19.37139351922690267, -277.1475549607477546, -316.7169759195553524 ) ) ;
#47575=CARTESIAN_POINT ( 'NONE',  ( -34.30880400572465305, -278.7746452029656439, -346.2872370499692352 ) ) ;
#47576=CARTESIAN_POINT ( 'NONE',  ( -64.52576852215828751, -275.4252178164295515, -340.6973120444997676 ) ) ;
#47577=CARTESIAN_POINT ( 'NONE',  ( -51.57958507967996553, -274.3575882932390186, -198.6484781452173252 ) ) ;
#47578=CARTESIAN_POINT ( 'NONE',  ( -94.90093830430885191, -295.7692264448830315, -224.5101744834705642 ) ) ;
#47580=CARTESIAN_POINT ( 'NONE',  ( -107.9731207818836936, -278.9629374276731824, -251.8674347539733844 ) ) ;
#47582=CARTESIAN_POINT ( 'NONE',  ( -59.89796240640044545, -288.0233021212309268, -343.4672962697396201 ) ) ;
#47583=CARTESIAN_POINT ( 'NONE',  ( 18.52851441622891215, -276.8548607413847549, -220.2496433184762168 ) ) ;
#47585=CARTESIAN_POINT ( 'NONE',  ( -95.08430858530101659, -289.1175331037509864, -315.3078900554295956 ) ) ;
#47586=CARTESIAN_POINT ( 'NONE',  ( -104.3322976382552980, -283.4089440004628386, -308.2257436787626261 ) ) ;
#47587=CARTESIAN_POINT ( 'NONE',  ( 30.23057755494690824, -280.1945898762396041, -300.6855665464400431 ) ) ;
#47588=CARTESIAN_POINT ( 'NONE',  ( 11.71198929502814501, -279.3240363667945871, -215.5057584475467252 ) ) ;
#47589=CARTESIAN_POINT ( 'NONE',  ( -90.67787887103109767, -283.3691259256360695, -218.3587014142066778 ) ) ;
#47590=CARTESIAN_POINT ( 'NONE',  ( -22.29675490276056848, -288.2448550826783276, -196.8331817600846705 ) ) ;
#47591=CARTESIAN_POINT ( 'NONE',  ( -110.5632759572167885, -279.6816070372574359, -276.1252648904854823 ) ) ;
#47593=CARTESIAN_POINT ( 'NONE',  ( -63.71014044453618652, -293.7087111566733029, -200.0945302020680856 ) ) ;
#47595=CARTESIAN_POINT ( 'NONE',  ( -111.4089096642188679, -277.0070971581349681, -253.3898926433860197 ) ) ;
#47596=CARTESIAN_POINT ( 'NONE',  ( -51.29222526829494910, -277.8866740735675762, -342.1195705589668137 ) ) ;
#47597=CARTESIAN_POINT ( 'NONE',  ( -91.10423642050577087, -285.8140612890744592, -322.8931854967257777 ) ) ;
#47599=CARTESIAN_POINT ( 'NONE',  ( -111.7581457573550523, -292.6392090248023123, -257.2650567603678269 ) ) ;
#47600=CARTESIAN_POINT ( 'NONE',  ( -85.33481484035438314, -293.7147043058071176, -328.0617980502964883 ) ) ;
#47601=CARTESIAN_POINT ( 'NONE',  ( 37.94801681810128002, -286.9416978265425655, -285.7109500091943914 ) ) ;
#47602=CARTESIAN_POINT ( 'NONE',  ( -109.4883952195729648, -289.1547155414114627, -254.8274511637614808 ) ) ;
#47603=CARTESIAN_POINT ( 'NONE',  ( 82.68073018288104947, -297.0543924324409204, -195.4120394483015559 ) ) ;
#47604=CARTESIAN_POINT ( 'NONE',  ( 1.115301559305689416, -275.2122857020949596, -333.0491960670415210 ) ) ;
#47605=CARTESIAN_POINT ( 'NONE',  ( 26.84905820180849645, -292.1948161928117429, -307.6493470018145899 ) ) ;
#47608=CARTESIAN_POINT ( 'NONE',  ( -19.52965614330108224, -290.7569505352001329, -196.1081412905921297 ) ) ;
#47609=CARTESIAN_POINT ( 'NONE',  ( -96.41845246222676735, -286.7663842029486432, -226.1301587960186623 ) ) ;
#47610=CARTESIAN_POINT ( 'NONE',  ( -37.52198627677552878, -287.2942095360349413, -346.3604735338157639 ) ) ;
#47611=CARTESIAN_POINT ( 'NONE',  ( -86.13026583795144120, -286.7854615180390283, -215.2016999400666180 ) ) ;
#47613=CARTESIAN_POINT ( 'NONE',  ( 4.810073576419219954, -287.4403704319697113, -210.5008873459819938 ) ) ;
#47614=CARTESIAN_POINT ( 'NONE',  ( 36.70423329606516205, -295.3533101847598346, -256.3751768772215200 ) ) ;
#47615=CARTESIAN_POINT ( 'NONE',  ( -108.3912483775651907, -276.2992734078989088, -296.2296007827430344 ) ) ;
#47616=CARTESIAN_POINT ( 'NONE',  ( 39.53294640657126990, -275.8238315351299548, -265.4368990987728125 ) ) ;
#47617=CARTESIAN_POINT ( 'NONE',  ( -1.465605998608614291, -290.6039150269379547, -203.8613430214066966 ) ) ;
#47618=CARTESIAN_POINT ( 'NONE',  ( -98.57635774909127235, -279.1747062544077949, -223.6564873353267160 ) ) ;
#47619=CARTESIAN_POINT ( 'NONE',  ( -97.72442964321508896, -297.9311378339749581, -314.2665527876299052 ) ) ;
#47621=CARTESIAN_POINT ( 'NONE',  ( 82.61707336526248469, -302.0539871969763226, -195.3101965168185075 ) ) ;
#47622=CARTESIAN_POINT ( 'NONE',  ( -9.289759988345592134, -285.1115109857813081, -202.4186417087223333 ) ) ;
#47623=CARTESIAN_POINT ( 'NONE',  ( -110.3425317100750505, -276.8666151121439611, -256.8798691341774543 ) ) ;
#47624=CARTESIAN_POINT ( 'NONE',  ( 35.39792894632608977, -279.3172539828678964, -252.0869007789418106 ) ) ;
#47626=CARTESIAN_POINT ( 'NONE',  ( 15.56042246569386123, -273.2641615382976852, -215.3695442951176062 ) ) ;
#47627=CARTESIAN_POINT ( 'NONE',  ( 35.00873177644231760, -295.2552802114641963, -284.3655014811394608 ) ) ;
#47628=CARTESIAN_POINT ( 'NONE',  ( 20.84060621698269955, -279.7952161945113971, -220.3780411768001102 ) ) ;
#47629=CARTESIAN_POINT ( 'NONE',  ( -41.03914793408155504, -296.0410437592004769, -343.5156244233089637 ) ) ;
#47630=CARTESIAN_POINT ( 'NONE',  ( -113.1615712570140317, -297.7336866771927930, -280.9781290011997612 ) ) ;
#47631=CARTESIAN_POINT ( 'NONE',  ( -37.82038706130927608, -297.8793107173324870, -197.3626874284838095 ) ) ;
#47632=CARTESIAN_POINT ( 'NONE',  ( -93.17872728426682727, -293.2499372518411747, -220.2696827246394378 ) ) ;
#47633=CARTESIAN_POINT ( 'NONE',  ( -110.9266604951672832, -285.0056532324294949, -247.5044796652495052 ) ) ;
#47634=CARTESIAN_POINT ( 'NONE',  ( 37.70401613017851616, -273.5593766588340259, -259.9473793853367738 ) ) ;
#47635=CARTESIAN_POINT ( 'NONE',  ( -54.50368079889251050, -289.0999634222840200, -345.4789130982442771 ) ) ;
#47637=CARTESIAN_POINT ( 'NONE',  ( 31.61693705707779145, -286.9381889639606129, -295.0211018719610365 ) ) ;
#47638=CARTESIAN_POINT ( 'NONE',  ( -94.12946154819205447, -289.2314237030576578, -221.3501623968813874 ) ) ;
#47640=CARTESIAN_POINT ( 'NONE',  ( 172.7732574597264659, 233.5132621949535121, -195.2123807395911399 ) ) ;
#47641=CARTESIAN_POINT ( 'NONE',  ( -13.27351186111235570, -288.2385630439052306, -339.3445272571921691 ) ) ;
#47643=CARTESIAN_POINT ( 'NONE',  ( -107.7152394915555789, -285.8870332966218371, -239.5624597823806141 ) ) ;
#47645=CARTESIAN_POINT ( 'NONE',  ( 19.25032963359218385, -291.9031308432815877, -218.4943426778026776 ) ) ;
#47646=CARTESIAN_POINT ( 'NONE',  ( 36.55044709686200122, -282.9169604685616264, -251.7495356683943157 ) ) ;
#47647=CARTESIAN_POINT ( 'NONE',  ( 23.34582961793901390, -282.2416224719971183, -223.7530071189453622 ) ) ;
#47648=CARTESIAN_POINT ( 'NONE',  ( -45.64157639274407785, -282.9934550536116262, -342.9387422208430962 ) ) ;
#47649=CARTESIAN_POINT ( 'NONE',  ( -35.03118515858106008, -279.0232862465290395, -345.3255240185489470 ) ) ;
#47650=CARTESIAN_POINT ( 'NONE',  ( -114.3097146207065578, -296.5974982793034087, -266.7352797015803390 ) ) ;
#47651=CARTESIAN_POINT ( 'NONE',  ( -92.88046569008872666, -289.2705273134654362, -220.4692463708019829 ) ) ;
#47653=CARTESIAN_POINT ( 'NONE',  ( -68.16500847693738763, -296.5579384447445364, -203.8331143420233218 ) ) ;
#47657=CARTESIAN_POINT ( 'NONE',  ( -95.25752081037309438, -287.1210467887561890, -223.5747658964220363 ) ) ;
#47658=CARTESIAN_POINT ( 'NONE',  ( 8.731465330671609237, -295.5166386557660871, -331.6698117666222743 ) ) ;
#47659=CARTESIAN_POINT ( 'NONE',  ( 9.980988713669042056, -283.0315010312393156, -326.1453366281459125 ) ) ;
#47660=CARTESIAN_POINT ( 'NONE',  ( -2.841629983217734967, -275.6661519946530916, -338.9510035292726684 ) ) ;
#47661=CARTESIAN_POINT ( 'NONE',  ( -47.73783457298037547, -292.5748200191452497, -194.1153131082313337 ) ) ;
#47662=CARTESIAN_POINT ( 'NONE',  ( -108.8042121782666669, -283.0144182493546055, -245.1933836623553589 ) ) ;
#47663=CARTESIAN_POINT ( 'NONE',  ( -81.92159288018133623, -291.7960432747566983, -207.6046246638865114 ) ) ;
#47664=CARTESIAN_POINT ( 'NONE',  ( -109.4393033478242074, -290.7317245770276486, -282.0165711778835771 ) ) ;
#47667=CARTESIAN_POINT ( 'NONE',  ( -109.6358133930788341, -268.7236802452458164, -295.3006767381334612 ) ) ;
#47668=CARTESIAN_POINT ( 'NONE',  ( -19.06552280945043876, -284.3413264348214398, -344.5012716072055241 ) ) ;
#47669=CARTESIAN_POINT ( 'NONE',  ( -110.4683760289727132, -281.8380690714489560, -287.0191576251351080 ) ) ;
#47671=CARTESIAN_POINT ( 'NONE',  ( 28.06336765206942729, -280.0234616424397132, -237.1365389942568527 ) ) ;
#47672=CARTESIAN_POINT ( 'NONE',  ( 37.21720677263221688, -275.4585890701054609, -289.5108880434040657 ) ) ;
#47673=CARTESIAN_POINT ( 'NONE',  ( -37.02551789679036176, -282.0562785194675826, -195.5284482456149533 ) ) ;
#47674=CARTESIAN_POINT ( 'NONE',  ( -61.30215766228251084, -183.8136707010272062, -360.3189382787912791 ) ) ;
#47675=CARTESIAN_POINT ( 'NONE',  ( 28.78580410112975230, -279.6251867241250011, -232.0758796252319769 ) ) ;
#47676=CARTESIAN_POINT ( 'NONE',  ( -110.2665141793495991, -282.7785645576452112, -254.3698580139528929 ) ) ;
#47677=CARTESIAN_POINT ( 'NONE',  ( 29.65232855243818832, -300.6400987876805857, -194.3546781410696269 ) ) ;
#47678=CARTESIAN_POINT ( 'NONE',  ( -12.98181965744049826, -295.2193703978383041, -339.2953684515639452 ) ) ;
#47680=CARTESIAN_POINT ( 'NONE',  ( 36.20138064381440302, -292.2424506577810348, -270.7793319094438402 ) ) ;
#47681=CARTESIAN_POINT ( 'NONE',  ( 5.820931290189878204, -277.1350206301834760, -334.0030855463894000 ) ) ;
#47682=CARTESIAN_POINT ( 'NONE',  ( -16.64066289968322465, -274.3270282708923560, -200.3050735678479555 ) ) ;
#47683=CARTESIAN_POINT ( 'NONE',  ( 25.80451277027892232, -275.0504242463206310, -313.9736759531064081 ) ) ;
#47685=CARTESIAN_POINT ( 'NONE',  ( -1.804745578269042694, -272.5227405973731152, -204.3004272533835888 ) ) ;
#47688=CARTESIAN_POINT ( 'NONE',  ( 17.84659108932734028, -283.3173887270186810, -318.6154295693416998 ) ) ;
#47689=CARTESIAN_POINT ( 'NONE',  ( 37.67115646527371808, -283.4669993684191240, -282.5687693303100900 ) ) ;
#47690=CARTESIAN_POINT ( 'NONE',  ( -100.4933566793570634, -283.3961040028550542, -307.1817771672111235 ) ) ;
#47691=CARTESIAN_POINT ( 'NONE',  ( 20.63845728254089806, -274.5893592052297549, -316.0404354382346241 ) ) ;
#47692=CARTESIAN_POINT ( 'NONE',  ( 20.32632437346097376, -284.0631475246072455, -317.1279740642792717 ) ) ;
#47693=CARTESIAN_POINT ( 'NONE',  ( -73.19611201322258864, -276.0165163483718516, -334.7586242900611637 ) ) ;
#47695=DIRECTION ( 'NONE',  ( 0.000000000000000000, 0.000000000000000000, 1.000000000000000000 ) ) ;
#47696=CARTESIAN_POINT ( 'NONE',  ( 34.42112294574901199, -276.4342778598795007, -255.3224628244218479 ) ) ;
#47699=CARTESIAN_POINT ( 'NONE',  ( -68.61618267290103290, -280.4543429325115085, -200.1608257721644861 ) ) ;
#47701=VERTEX_POINT ( 'NONE', #59398 ) ;
#47703=CARTESIAN_POINT ( 'NONE',  ( -54.70491745366501846, -287.6917080216013574, -196.6127338519378043 ) ) ;
#47704=CARTESIAN_POINT ( 'NONE',  ( 6.150742960839347795, -293.6422031563332666, -329.2545890534848354 ) ) ;
#47705=CARTESIAN_POINT ( 'NONE',  ( -97.21594565599330906, -289.2528314534004039, -318.6352542560511552 ) ) ;
#47706=CARTESIAN_POINT ( 'NONE',  ( 34.68207832655853906, -286.0138037230846066, -287.4066262950659052 ) ) ;
#47707=CARTESIAN_POINT ( 'NONE',  ( -22.32197938764292999, -284.8228513987478436, -198.2686678903622806 ) ) ;
#47708=CARTESIAN_POINT ( 'NONE',  ( -110.2714042347649297, -288.9599911570866198, -257.4502746748822233 ) ) ;
#47709=CARTESIAN_POINT ( 'NONE',  ( -110.4902457411891703, -285.6780536511303126, -276.3960810136822488 ) ) ;
#47710=CARTESIAN_POINT ( 'NONE',  ( -3.647065475366475074, -274.6074148424914370, -337.3804293146052373 ) ) ;
#47711=CARTESIAN_POINT ( 'NONE',  ( -60.24979907409539237, -284.1600202365473251, -197.6310987883229586 ) ) ;
#47712=CARTESIAN_POINT ( 'NONE',  ( -23.83641044767545836, -300.2213687122415422, -195.3565049566856828 ) ) ;
#47713=CARTESIAN_POINT ( 'NONE',  ( 34.11436224735621892, -285.2494619235554296, -246.8693992218734365 ) ) ;
#47714=CARTESIAN_POINT ( 'NONE',  ( 33.98684027382742556, -282.2750893985226526, -253.7584744255732687 ) ) ;
#47715=CARTESIAN_POINT ( 'NONE',  ( -64.75411163116002911, -291.4093006804125139, -340.4060248311345163 ) ) ;
#47718=CARTESIAN_POINT ( 'NONE',  ( -68.90371440078584442, -297.3840149352756725, -339.0276890524650639 ) ) ;
#47719=CARTESIAN_POINT ( 'NONE',  ( -96.34901561848397478, -277.1875605739548973, -224.0464252348748744 ) ) ;
#47720=CARTESIAN_POINT ( 'NONE',  ( -25.03720412211271906, -291.4024283152998578, -194.5141787027797307 ) ) ;
#47721=CARTESIAN_POINT ( 'NONE',  ( -111.0096578522765896, -295.0095970857670409, -265.9483616804477606 ) ) ;
#47722=CARTESIAN_POINT ( 'NONE',  ( 33.42984690800979308, -280.4971180891677704, -290.1760519707942763 ) ) ;
#47723=CARTESIAN_POINT ( 'NONE',  ( -0.9986393045823697134, -272.6183191392937033, -205.3811743587416174 ) ) ;
#47724=CARTESIAN_POINT ( 'NONE',  ( 11.24436098399135098, -294.0568811471003414, -215.1512425903901544 ) ) ;
#47725=CARTESIAN_POINT ( 'NONE',  ( -106.6662871844225293, -293.4805209788415823, -237.0123917617630696 ) ) ;
#47726=CARTESIAN_POINT ( 'NONE',  ( -113.6157599027163627, -295.0776209862428914, -266.7486222704873171 ) ) ;
#47727=CARTESIAN_POINT ( 'NONE',  ( 38.64354924975474148, -291.7557191225909605, -267.4974502809838555 ) ) ;
#47728=CARTESIAN_POINT ( 'NONE',  ( -95.59184054737738734, -292.6054652558211160, -225.3911717963164278 ) ) ;
#47730=CARTESIAN_POINT ( 'NONE',  ( -75.07162759039111677, -292.3387569462754527, -207.6197985925956857 ) ) ;
#47732=CARTESIAN_POINT ( 'NONE',  ( -104.3337067412666812, -282.1165640111130415, -304.9783448220904916 ) ) ;
#47733=CARTESIAN_POINT ( 'NONE',  ( -20.07216374514698742, -292.2801834026947745, -199.3809759998275410 ) ) ;
#47734=CARTESIAN_POINT ( 'NONE',  ( 36.98501116077425621, -281.2997050018714731, -250.1979371213774925 ) ) ;
#47735=CARTESIAN_POINT ( 'NONE',  ( -109.2847105019817349, -283.8704616686964641, -297.8948449141982451 ) ) ;
#47736=CARTESIAN_POINT ( 'NONE',  ( -64.50965489499087369, -287.4072960804297168, -340.1442181516828782 ) ) ;
#47738=CARTESIAN_POINT ( 'NONE',  ( -39.54764277663036864, -278.5048414751907444, -194.0734077914263764 ) ) ;
#47739=CARTESIAN_POINT ( 'NONE',  ( 39.39296711314005250, -286.4875392341477891, -271.5602332263627545 ) ) ;
#47741=CARTESIAN_POINT ( 'NONE',  ( 34.07730842769990431, -294.9094495733689882, -251.7663436137316353 ) ) ;
#47742=CARTESIAN_POINT ( 'NONE',  ( 10.17395498617785599, -277.8371215589682492, -330.2690562992742684 ) ) ;
#47743=CARTESIAN_POINT ( 'NONE',  ( -93.95423220729134073, -278.8715256370971360, -224.2405293213952291 ) ) ;
#47744=CARTESIAN_POINT ( 'NONE',  ( 28.05123619982690997, -293.1858820149072358, -229.6061752685889985 ) ) ;
#47745=CARTESIAN_POINT ( 'NONE',  ( -38.73105522070399331, -281.1493020782292547, -345.9083475415899329 ) ) ;
#47746=CARTESIAN_POINT ( 'NONE',  ( 33.67128884787867804, -292.8464354397736997, -288.2654148269921848 ) ) ;
#47747=CARTESIAN_POINT ( 'NONE',  ( -112.1244148901376150, -294.6334884768492657, -264.0136916087113264 ) ) ;
#47750=CARTESIAN_POINT ( 'NONE',  ( 34.89785664870981918, -293.2081829504113557, -281.6186346569671173 ) ) ;
#47752=CARTESIAN_POINT ( 'NONE',  ( 7.399455738971487229, -285.9094976428776249, -326.5171145203363494 ) ) ;
#47753=CARTESIAN_POINT ( 'NONE',  ( -26.23994229802980271, -297.2467105780751240, -193.5981341315722659 ) ) ;
#47754=CARTESIAN_POINT ( 'NONE',  ( 3.181661219328753454, -278.7294789342200261, -206.2822416791846081 ) ) ;
#47755=CARTESIAN_POINT ( 'NONE',  ( -4.997753247498134321, -287.7843169035766664, -201.0273789015625425 ) ) ;
#47756=CARTESIAN_POINT ( 'NONE',  ( 29.42419740904362158, -287.7842185941754565, -300.0045690794859752 ) ) ;
#47757=CARTESIAN_POINT ( 'NONE',  ( -29.62172352023252486, -278.4728987251283456, -343.7003633859345655 ) ) ;
#47758=CARTESIAN_POINT ( 'NONE',  ( -104.2535083699871450, -294.1322979533326247, -303.5635983049475044 ) ) ;
#47759=CARTESIAN_POINT ( 'NONE',  ( -50.15102219760230184, -299.6465829423858054, -197.4646483878504455 ) ) ;
#47760=CARTESIAN_POINT ( 'NONE',  ( -109.1564520441392148, -277.1481934026274416, -285.5193472089760007 ) ) ;
#47762=CARTESIAN_POINT ( 'NONE',  ( -30.48266029254661547, -297.8025502153051889, -193.3826370686200846 ) ) ;
#47763=CARTESIAN_POINT ( 'NONE',  ( -50.99199153367960946, -291.1479538660603339, -343.5915674354181419 ) ) ;
#47764=CARTESIAN_POINT ( 'NONE',  ( 25.07123255647881876, -295.7366338377801185, -314.0996418343348182 ) ) ;
#47765=CARTESIAN_POINT ( 'NONE',  ( 202.0868887437326009, 292.1662959946771139, -53.99999999997601918 ) ) ;
#47766=CARTESIAN_POINT ( 'NONE',  ( -102.5041869584556196, -291.6542605405141444, -237.1168346312996391 ) ) ;
#47768=CARTESIAN_POINT ( 'NONE',  ( -98.15846494899039953, -297.8328633425223870, -223.2799665494169687 ) ) ;
#47769=CARTESIAN_POINT ( 'NONE',  ( -91.90580513875376312, -289.4238143662906850, -217.7216511321033181 ) ) ;
#47770=CARTESIAN_POINT ( 'NONE',  ( -14.82206327796470013, -298.6601616315489878, -193.3810252821741074 ) ) ;
#47772=CARTESIAN_POINT ( 'NONE',  ( -36.07872676323889749, -290.5567359591474883, -346.6703265333196669 ) ) ;
#47773=CARTESIAN_POINT ( 'NONE',  ( -55.56934967048406548, -279.7662352645559736, -350.3683826091709648 ) ) ;
#47774=CARTESIAN_POINT ( 'NONE',  ( -88.97748520626691970, -287.3245327908676359, -216.1967927859187455 ) ) ;
#47775=CARTESIAN_POINT ( 'NONE',  ( 13.86557104076155689, -285.3281008006022716, -213.5766099432649980 ) ) ;
#47776=CARTESIAN_POINT ( 'NONE',  ( 35.29469311191165559, -273.3202936069629345, -252.3615955638833839 ) ) ;
#47777=CARTESIAN_POINT ( 'NONE',  ( -49.12706271512227119, -275.8211213865592981, -196.8077806674050976 ) ) ;
#47778=CARTESIAN_POINT ( 'NONE',  ( -111.0522243948232557, -288.4963238075204117, -280.8485848479246556 ) ) ;
#47779=CARTESIAN_POINT ( 'NONE',  ( -35.71390687493809679, -278.8923790394271691, -346.1213460299987332 ) ) ;
#47781=ORIENTED_EDGE ( 'NONE', *, *, #12669, .F. ) ;
#47782=CARTESIAN_POINT ( 'NONE',  ( -11.74314832479123893, -280.3948230826503050, -201.9430927547477950 ) ) ;
#47783=CARTESIAN_POINT ( 'NONE',  ( -9.200451133116812841, -279.7786682168504626, -202.8928826909244378 ) ) ;
#47784=CARTESIAN_POINT ( 'NONE',  ( -14.66790997642876704, -277.8448258570442135, -343.6792079792042500 ) ) ;
#47785=CARTESIAN_POINT ( 'NONE',  ( 28.95067408403298970, -279.8453478236557430, -231.9771390454549476 ) ) ;
#47786=CARTESIAN_POINT ( 'NONE',  ( -14.03755197167841295, -91.47614451431806515, -356.9296174414798770 ) ) ;
#47787=CARTESIAN_POINT ( 'NONE',  ( 25.12842388375779734, -275.9003647540504858, -225.7258142996655295 ) ) ;
#47788=CARTESIAN_POINT ( 'NONE',  ( -99.01819550539553916, -274.6749868029116328, -225.3433311945190667 ) ) ;
#47789=CARTESIAN_POINT ( 'NONE',  ( -20.19161114001083490, -297.3376638359846424, -345.3538533559490702 ) ) ;
#47792=CARTESIAN_POINT ( 'NONE',  ( 27.92711316866997251, -288.1788801405559752, -236.8694787884889479 ) ) ;
#47793=CARTESIAN_POINT ( 'NONE',  ( 18.88966181576476799, -290.0162628869611581, -321.4883127545409707 ) ) ;
#47794=CARTESIAN_POINT ( 'NONE',  ( -97.43742830510288400, -289.3213908267341026, -312.0051761180399694 ) ) ;
#47795=CARTESIAN_POINT ( 'NONE',  ( 23.81633760228273289, -286.4366923169906158, -223.6573842876974254 ) ) ;
#47797=CARTESIAN_POINT ( 'NONE',  ( 14.47199614912897836, -280.7087026063785515, -322.9857025533169121 ) ) ;
#47798=CARTESIAN_POINT ( 'NONE',  ( 18.77455666692207714, -290.0942689705481712, -319.0367886127818338 ) ) ;
#47799=CARTESIAN_POINT ( 'NONE',  ( -8.238070374407035601, -281.1438298552202468, -338.0640461972238882 ) ) ;
#47801=CARTESIAN_POINT ( 'NONE',  ( -108.9631019788419479, -279.6506469371350363, -286.8976813401220056 ) ) ;
#47802=CARTESIAN_POINT ( 'NONE',  ( 19.23322490027285525, -276.6987228228639424, -316.6114121402917476 ) ) ;
#47803=CARTESIAN_POINT ( 'NONE',  ( -101.3437162637597027, -289.9043805502423652, -228.1737897792467322 ) ) ;
#47804=CARTESIAN_POINT ( 'NONE',  ( -112.2047216655330857, -285.5719406928964759, -253.0496527733878622 ) ) ;
#47805=CARTESIAN_POINT ( 'NONE',  ( -52.16757244290418072, -286.3597199234480968, -194.8102777431788297 ) ) ;
#47806=CARTESIAN_POINT ( 'NONE',  ( 33.11302353964201473, -281.4658421557255110, -251.2048732497125343 ) ) ;
#47809=CARTESIAN_POINT ( 'NONE',  ( -99.65106335666747839, -291.8340225229222256, -313.4638874422210506 ) ) ;
#47810=CARTESIAN_POINT ( 'NONE',  ( -25.08384501134178990, -290.8901693776799107, -194.8426218403851067 ) ) ;
#47811=CARTESIAN_POINT ( 'NONE',  ( 13.66911008037368269, -273.8473572301384706, -217.8129906166182934 ) ) ;
#47812=CARTESIAN_POINT ( 'NONE',  ( -16.54243468085542901, -294.1389688019206687, -344.4480482461646034 ) ) ;
#47813=CARTESIAN_POINT ( 'NONE',  ( -69.30093676245908796, -290.1037844213788048, -203.9445123520838479 ) ) ;
#47814=CARTESIAN_POINT ( 'NONE',  ( -20.64101670490907736, -293.0747841058794165, -342.5184576341039246 ) ) ;
#47815=CARTESIAN_POINT ( 'NONE',  ( -109.6707149694501169, -291.9247291296268827, -257.5948483605287720 ) ) ;
#47817=CARTESIAN_POINT ( 'NONE',  ( -110.6060244640538741, -292.3463345844836567, -286.4029206480037715 ) ) ;
#47818=CARTESIAN_POINT ( 'NONE',  ( -22.52952526021267587, -290.2410455688940374, -196.6152882260547301 ) ) ;
#47819=CARTESIAN_POINT ( 'NONE',  ( 11.45536953088858745, -296.3760993425053698, -327.3835223753573018 ) ) ;
#47820=CARTESIAN_POINT ( 'NONE',  ( 9.170723964078902668, -287.6506648680766602, -213.7925502753100773 ) ) ;
#47821=CARTESIAN_POINT ( 'NONE',  ( 35.68509231518050484, -295.7811210911065132, -288.2228034533956702 ) ) ;
#47822=CARTESIAN_POINT ( 'NONE',  ( -32.80731966488770013, -276.0888882189502738, -195.1295922292562182 ) ) ;
#47823=CARTESIAN_POINT ( 'NONE',  ( 19.57185407617239292, -275.0468724302438659, -321.6531149912864294 ) ) ;
#47824=CARTESIAN_POINT ( 'NONE',  ( -89.49119200185317879, -296.5370042798498957, -213.8568853697558723 ) ) ;
#47825=CARTESIAN_POINT ( 'NONE',  ( 24.82349123551642478, -274.3416146429535161, -310.6235094109042620 ) ) ;
#47826=CARTESIAN_POINT ( 'NONE',  ( 10.21492164000678748, -278.7933868655203469, -213.0253975684684917 ) ) ;
#47827=CARTESIAN_POINT ( 'NONE',  ( -102.3894274533558786, -274.2187119351623323, -236.2521164373142142 ) ) ;
#47828=CARTESIAN_POINT ( 'NONE',  ( -0.3149494975562946997, -273.1092464090923499, -203.5059354400994209 ) ) ;
#47829=CARTESIAN_POINT ( 'NONE',  ( -107.4249011044205275, -297.6802210614119417, -292.9696548112023038 ) ) ;
#47831=CARTESIAN_POINT ( 'NONE',  ( -70.54996040007995362, -298.4055021964833827, -205.1565836681555481 ) ) ;
#47833=CARTESIAN_POINT ( 'NONE',  ( 2.293104917632814654, -286.5445401989034053, -334.5120132109231577 ) ) ;
#47834=CARTESIAN_POINT ( 'NONE',  ( -106.3056896592338632, -272.7038119997216086, -246.4243648099739232 ) ) ;
#47835=CARTESIAN_POINT ( 'NONE',  ( 38.97527028884086775, -287.4241708756740650, -260.1278376491272866 ) ) ;
#47836=CARTESIAN_POINT ( 'NONE',  ( -8.245058753504640237, -288.3481472887648920, -341.6433934503226055 ) ) ;
#47837=CARTESIAN_POINT ( 'NONE',  ( -96.94876041265688116, -299.1611270003007803, -224.2381665219304807 ) ) ;
#47838=CARTESIAN_POINT ( 'NONE',  ( -68.07075690856088102, -293.4563744284378686, -338.6082530300341205 ) ) ;
#47839=CARTESIAN_POINT ( 'NONE',  ( 3.744286426782932331, -279.7868918598464347, -205.3667571429196812 ) ) ;
#47841=CARTESIAN_POINT ( 'NONE',  ( -97.17354021324520374, -277.1706422857423604, -225.1168075251522964 ) ) ;
#47843=CARTESIAN_POINT ( 'NONE',  ( -58.81990368103672751, -288.1310301383136334, -340.5983800547072633 ) ) ;
#47846=CARTESIAN_POINT ( 'NONE',  ( -102.8587301140240982, -289.0390828466231596, -233.7508212618621144 ) ) ;
#47847=CARTESIAN_POINT ( 'NONE',  ( -110.8820953015494268, -274.1438931321728205, -264.8809920944484588 ) ) ;
#47848=CARTESIAN_POINT ( 'NONE',  ( 15.36035717930338862, -283.7500232587835285, -325.6883214846540682 ) ) ;
#47849=CARTESIAN_POINT ( 'NONE',  ( -105.5329531306852715, -271.0572056691246985, -237.8147324832247023 ) ) ;
#47850=CARTESIAN_POINT ( 'NONE',  ( -92.55912865390867239, -283.8716113710611921, -318.1298587852643323 ) ) ;
#47851=CARTESIAN_POINT ( 'NONE',  ( -6.296779724573521975, -275.8934980145440363, -203.6408973889737979 ) ) ;
#47852=CARTESIAN_POINT ( 'NONE',  ( 34.99978909241605862, -276.2101060891602060, -259.3539608691125409 ) ) ;
#47853=CARTESIAN_POINT ( 'NONE',  ( -41.43385859670913618, -285.1037115942406786, -345.3003689542235861 ) ) ;
#47854=CARTESIAN_POINT ( 'NONE',  ( -107.4882964293772147, -271.7553894491489928, -248.8875465601180395 ) ) ;
#47857=CARTESIAN_POINT ( 'NONE',  ( 37.08313043890141358, -293.1376742429494584, -250.5632276277583514 ) ) ;
#47858=CARTESIAN_POINT ( 'NONE',  ( -111.6340153215883646, -286.6321279601000924, -262.6036241156826350 ) ) ;
#47860=CARTESIAN_POINT ( 'NONE',  ( 25.22466315766302358, -278.4094976428775681, -220.5068182859052968 ) ) ;
#47861=CARTESIAN_POINT ( 'NONE',  ( -45.64235679010576519, -276.3518492002178277, -346.8029253531821041 ) ) ;
#47862=CARTESIAN_POINT ( 'NONE',  ( -112.3806290127888019, -289.1194952750862512, -257.1097192530816073 ) ) ;
#47863=CARTESIAN_POINT ( 'NONE',  ( 10.37220342581547250, -283.9000699950152580, -326.5895365445584275 ) ) ;
#47864=CARTESIAN_POINT ( 'NONE',  ( -21.41339368267877319, -278.6053847980942919, -342.6928996487774270 ) ) ;
#47865=CARTESIAN_POINT ( 'NONE',  ( -33.07337690516038009, -284.4246778165598357, -346.6656178578430172 ) ) ;
#47866=CARTESIAN_POINT ( 'NONE',  ( -16.03179388071970735, -281.5652572259400586, -340.5965677191549617 ) ) ;
#47867=CARTESIAN_POINT ( 'NONE',  ( -77.92492234900896619, -281.5074748229842498, -207.2277857257063829 ) ) ;
#47868=CARTESIAN_POINT ( 'NONE',  ( 23.63154151060813746, -275.0910173866198534, -223.3155802605577946 ) ) ;
#47869=CARTESIAN_POINT ( 'NONE',  ( -59.66703806442128410, -277.1668859834958312, -344.0535822548152396 ) ) ;
#47871=CARTESIAN_POINT ( 'NONE',  ( -109.3565713551685974, -298.2277058942799499, -289.2574722428213363 ) ) ;
#47874=CARTESIAN_POINT ( 'NONE',  ( -103.5354707400467049, -294.2048701747056612, -307.3288421930412824 ) ) ;
#47875=CARTESIAN_POINT ( 'NONE',  ( 19.22525981777495829, -275.7141878156453458, -316.6211532478974959 ) ) ;
#47876=CARTESIAN_POINT ( 'NONE',  ( 19.09207634808648280, -299.8228228643003490, -193.6601402860643759 ) ) ;
#47877=CARTESIAN_POINT ( 'NONE',  ( 27.24079331655068259, -288.8232758816945420, -234.1028129773707178 ) ) ;
#47878=CARTESIAN_POINT ( 'NONE',  ( -76.70780334520587473, -297.0887118748589160, -335.7909046014019054 ) ) ;
#47879=CARTESIAN_POINT ( 'NONE',  ( 37.07793189106546805, -294.9861650061301930, -288.5744393602686273 ) ) ;
#47880=CARTESIAN_POINT ( 'NONE',  ( -95.51375768354770912, -291.9027365835846695, -317.4359536251132567 ) ) ;
#47881=CARTESIAN_POINT ( 'NONE',  ( -94.47378737337868415, -277.2222716851174482, -222.0097174547422298 ) ) ;
#47882=CARTESIAN_POINT ( 'NONE',  ( -111.5967618395086021, -280.5401514404231875, -265.1170731771273950 ) ) ;
#47883=CARTESIAN_POINT ( 'NONE',  ( -111.5366246619025929, -294.5460533690520037, -277.0042905862908356 ) ) ;
#47884=CARTESIAN_POINT ( 'NONE',  ( 3.893629279626806827, -284.3641351983017671, -333.9837616488585468 ) ) ;
#47885=CARTESIAN_POINT ( 'NONE',  ( 0.3392986430308853052, -285.4868086662958149, -207.4181615756862413 ) ) ;
#47886=CARTESIAN_POINT ( 'NONE',  ( -110.6519398798504454, -271.9518965266826740, -296.2779929517423625 ) ) ;
#47888=CARTESIAN_POINT ( 'NONE',  ( -94.13580901942997059, -284.8679763692716165, -224.4444974290897790 ) ) ;
#47891=CARTESIAN_POINT ( 'NONE',  ( 9.032857052580727242, -283.5118974878466247, -331.4421539527042455 ) ) ;
#47892=CARTESIAN_POINT ( 'NONE',  ( -69.50409694271554883, -273.9499993768540094, -204.8045186350234133 ) ) ;
#47893=CARTESIAN_POINT ( 'NONE',  ( -35.14417093109853596, -284.8740661733422144, -193.7766406045116980 ) ) ;
#47894=CARTESIAN_POINT ( 'NONE',  ( 6.041379444771633800, -281.5664161416378306, -207.0308043942508505 ) ) ;
#47897=CARTESIAN_POINT ( 'NONE',  ( -68.40813783438576934, -281.1715163391167494, -200.6504883552492231 ) ) ;
#47898=CARTESIAN_POINT ( 'NONE',  ( 20.11007591016628382, -281.1904247046184082, -219.1061771533815943 ) ) ;
#47899=CARTESIAN_POINT ( 'NONE',  ( 17.36665895637873192, -279.6952119285918457, -314.0302885647153062 ) ) ;
#47900=CARTESIAN_POINT ( 'NONE',  ( 162.1785412711766128, 219.9095514846544290, -205.3156639783633750 ) ) ;
#47902=CARTESIAN_POINT ( 'NONE',  ( -10.86481649574293229, -276.3981916849856475, -200.3128440212580301 ) ) ;
#47903=CARTESIAN_POINT ( 'NONE',  ( -22.71367860124261639, -107.9710121992093548, -362.4982422966238573 ) ) ;
#47904=CARTESIAN_POINT ( 'NONE',  ( -1.146933343844307229, -278.5550833281416203, -205.0787646125536696 ) ) ;
#47905=CARTESIAN_POINT ( 'NONE',  ( -19.64482113742459291, -294.0366858884390808, -196.4098327872376899 ) ) ;
#47906=CARTESIAN_POINT ( 'NONE',  ( -18.20178933767734719, -294.1474459971979059, -340.9129179794224456 ) ) ;
#47907=CARTESIAN_POINT ( 'NONE',  ( -3.342891669507786823, -291.9966977106649324, -201.3276957806842802 ) ) ;
#47909=CARTESIAN_POINT ( 'NONE',  ( -81.54573278372066625, -294.2150394297707408, -332.7523903131476573 ) ) ;
#47910=CARTESIAN_POINT ( 'NONE',  ( 33.80588292249433380, -285.6957415018386541, -250.7534194303607364 ) ) ;
#47911=CARTESIAN_POINT ( 'NONE',  ( 36.65756893977778219, -295.4892897801606182, -276.2749708596793425 ) ) ;
#47912=CARTESIAN_POINT ( 'NONE',  ( -93.79016869040778204, -285.2039898738940451, -317.4229270886758059 ) ) ;
#47914=CARTESIAN_POINT ( 'NONE',  ( -81.80388354382461102, -292.4039162023991594, -207.7836902768522691 ) ) ;
#47915=CARTESIAN_POINT ( 'NONE',  ( -18.71389996809472223, -283.2982057526010635, -341.0605314025556822 ) ) ;
#47916=CARTESIAN_POINT ( 'NONE',  ( -111.2349347311150467, -295.6035471771603511, -249.9712368565271845 ) ) ;
#47917=CARTESIAN_POINT ( 'NONE',  ( -99.90552625284237820, -291.9470480884953076, -225.7525259700396987 ) ) ;
#47918=CARTESIAN_POINT ( 'NONE',  ( -61.67506738337655037, -292.2367252449123498, -197.3158671677418567 ) ) ;
#47919=CARTESIAN_POINT ( 'NONE',  ( 19.51482190470161626, -288.3661586537534731, -316.1468789446202550 ) ) ;
#47922=CARTESIAN_POINT ( 'NONE',  ( -108.2726552023081581, -298.0685278649633005, -297.1380371930032425 ) ) ;
#47923=CARTESIAN_POINT ( 'NONE',  ( -87.12856187305669664, -296.0606127347402889, -212.2002718345608230 ) ) ;
#47925=CARTESIAN_POINT ( 'NONE',  ( -49.16813861137797659, -278.9564720564790150, -198.0870299540867734 ) ) ;
#47926=CARTESIAN_POINT ( 'NONE',  ( 38.15957044152528965, -274.8745458836051512, -255.5595962432047941 ) ) ;
#47927=CARTESIAN_POINT ( 'NONE',  ( -109.4536042943176142, -295.2312333953454981, -255.1156266051811201 ) ) ;
#47928=CARTESIAN_POINT ( 'NONE',  ( -85.89553235068845538, -279.5931342318965562, -326.5842523410223635 ) ) ;
#47929=CARTESIAN_POINT ( 'NONE',  ( 35.04339195995451917, -273.4774186380431615, -253.8341104500827612 ) ) ;
#47930=CARTESIAN_POINT ( 'NONE',  ( -61.12741337681901399, -296.5728920410757041, -339.8510678751912337 ) ) ;
#47931=CARTESIAN_POINT ( 'NONE',  ( -108.4782262616793105, -297.8652225752066443, -252.5946998227687175 ) ) ;
#47933=CARTESIAN_POINT ( 'NONE',  ( -108.1528092270744565, -298.5146699405961499, -242.0726934031937674 ) ) ;
#47934=CARTESIAN_POINT ( 'NONE',  ( -54.15960630100301643, -295.8364965095256593, -197.1000338014080739 ) ) ;
#47935=CARTESIAN_POINT ( 'NONE',  ( 10.99199535900419100, -293.3932271740039823, -215.4506523899968897 ) ) ;
#47936=CARTESIAN_POINT ( 'NONE',  ( -108.9277979490158543, -288.9037021465399562, -287.4141387637314438 ) ) ;
#47938=CARTESIAN_POINT ( 'NONE',  ( 7.194257009148517845, -275.1330625948261286, -207.5575897496810001 ) ) ;
#47939=CARTESIAN_POINT ( 'NONE',  ( -76.56601569282112507, -273.6778074237018927, -208.7944624539895244 ) ) ;
#47940=CARTESIAN_POINT ( 'NONE',  ( 5.233733975371583469, -282.6048890810330363, -208.1860489321172167 ) ) ;
#47941=CARTESIAN_POINT ( 'NONE',  ( 22.12928338929965832, -280.8867588966585345, -318.5118181721572341 ) ) ;
#47943=CARTESIAN_POINT ( 'NONE',  ( -72.80106846456230585, -276.8578910992707733, -338.6102955469083327 ) ) ;
#47944=CARTESIAN_POINT ( 'NONE',  ( -110.1540600138141315, -283.8498515584774395, -262.7230530015149839 ) ) ;
#47945=CARTESIAN_POINT ( 'NONE',  ( 20.18997449898513707, -280.2192876561621233, -318.7360582357040357 ) ) ;
#47946=CARTESIAN_POINT ( 'NONE',  ( -68.51580212926013758, -272.2090690184517143, -203.6873507035834621 ) ) ;
#47947=CARTESIAN_POINT ( 'NONE',  ( -29.51147819262562066, -278.9532711824034550, -345.0022699460427589 ) ) ;
#47950=CARTESIAN_POINT ( 'NONE',  ( 74.55052467484399870, -297.6744934986045905, -194.4074022689418086 ) ) ;
#47951=CARTESIAN_POINT ( 'NONE',  ( -4.765771754016490114, -278.6242992926111697, -338.1162318610784041 ) ) ;
#47952=CARTESIAN_POINT ( 'NONE',  ( -29.76311809300124978, -272.1479549999277197, -195.7449954456092485 ) ) ;
#47954=CARTESIAN_POINT ( 'NONE',  ( -111.1137661218266288, -286.2640516088807772, -286.7011449547217126 ) ) ;
#47957=CARTESIAN_POINT ( 'NONE',  ( 20.22899615849963695, -286.2161809148599332, -318.4496845795161448 ) ) ;
#47959=CARTESIAN_POINT ( 'NONE',  ( -37.00907922970003483, -293.8427857833765415, -343.7699299751866988 ) ) ;
#47960=CARTESIAN_POINT ( 'NONE',  ( 25.26760187291327142, -286.2340869954373375, -310.2477170166627616 ) ) ;
#47961=CARTESIAN_POINT ( 'NONE',  ( 201.7194887906492795, 294.2213704821156739, -83.28174295417332473 ) ) ;
#47962=CARTESIAN_POINT ( 'NONE',  ( -100.4290682116322841, -294.0045845161777720, -311.0147151388366638 ) ) ;
#47963=CARTESIAN_POINT ( 'NONE',  ( -10.22210209114956569, -284.8795340388236923, -198.9799659732566965 ) ) ;
#47964=CARTESIAN_POINT ( 'NONE',  ( 3.125813926382862817, -282.2053889370845354, -208.5841649242665596 ) ) ;
#47965=CARTESIAN_POINT ( 'NONE',  ( 16.52085195812075469, -279.0444582799065643, -216.6888108236538812 ) ) ;
#47966=CARTESIAN_POINT ( 'NONE',  ( 17.82553026358253945, -288.2341536596968581, -318.2445072733001439 ) ) ;
#47967=CARTESIAN_POINT ( 'NONE',  ( -110.2078586681560068, -280.1167286527313536, -259.7162629346179301 ) ) ;
#47968=CARTESIAN_POINT ( 'NONE',  ( -76.91778337390783804, -280.3103398369945580, -208.7675153864627191 ) ) ;
#47969=CARTESIAN_POINT ( 'NONE',  ( 36.93130988676805515, -289.3684563766395286, -257.5603081369066558 ) ) ;
#47971=CARTESIAN_POINT ( 'NONE',  ( -49.71923897398222891, -273.8985981582165437, -194.3086511941902472 ) ) ;
#47972=CARTESIAN_POINT ( 'NONE',  ( -83.54504528438066302, -291.6693604290020403, -328.9878840192811822 ) ) ;
#47974=CARTESIAN_POINT ( 'NONE',  ( -88.47809603358389552, -292.1948066931273615, -334.5364918783848793 ) ) ;
#47976=CARTESIAN_POINT ( 'NONE',  ( 34.83287086736124394, -273.2801550703312614, -249.1823495373240576 ) ) ;
#47978=CARTESIAN_POINT ( 'NONE',  ( -37.70582191463291366, -293.4564829181189793, -346.5731929530072648 ) ) ;
#47979=CARTESIAN_POINT ( 'NONE',  ( -110.4433243138642950, -271.9367760107406866, -267.6251805984415455 ) ) ;
#47980=CARTESIAN_POINT ( 'NONE',  ( -0.6293907000458592860, -290.0754301642651285, -334.3175481656742818 ) ) ;
#47981=CARTESIAN_POINT ( 'NONE',  ( -37.52077331648934688, -284.8146010123085716, -344.3868395776810871 ) ) ;
#47982=CARTESIAN_POINT ( 'NONE',  ( -96.81989079904772666, -291.3291805808991626, -318.3499770783621443 ) ) ;
#47983=CARTESIAN_POINT ( 'NONE',  ( -111.8409139349781753, -292.0864858177499741, -252.9494719604173270 ) ) ;
#47984=CARTESIAN_POINT ( 'NONE',  ( -33.15171718094730835, -288.1049510643959479, -195.4270590555443334 ) ) ;
#47985=CARTESIAN_POINT ( 'NONE',  ( -99.42912640366540700, -279.3239181208564332, -224.7960109422399171 ) ) ;
#47986=CARTESIAN_POINT ( 'NONE',  ( -112.2289013216337707, -294.4988804527592379, -280.8061139300600644 ) ) ;
#47987=CARTESIAN_POINT ( 'NONE',  ( -5.457456127174665994, -282.4774799173404745, -340.4495976994124931 ) ) ;
#47988=CARTESIAN_POINT ( 'NONE',  ( 8.068106416014980908, -276.5409992106419281, -211.6345060669696636 ) ) ;
#47989=CARTESIAN_POINT ( 'NONE',  ( -67.68488546085839630, -279.9805209788415823, -333.4427485647536855 ) ) ;
#47990=CARTESIAN_POINT ( 'NONE',  ( 21.98149345425066770, -273.1473032778117158, -222.8564501972736878 ) ) ;
#47992=CARTESIAN_POINT ( 'NONE',  ( 4.963885067016563291, -280.1490989473991249, -210.7941312970201579 ) ) ;
#47993=CARTESIAN_POINT ( 'NONE',  ( -67.53788651524465081, -278.6446593559310827, -340.7613953044958066 ) ) ;
#47994=CARTESIAN_POINT ( 'NONE',  ( -43.63498782813222476, -285.0333618627391843, -193.8017165078334756 ) ) ;
#47995=CARTESIAN_POINT ( 'NONE',  ( -69.47758036835661244, -293.3835163385631972, -203.6743444191989454 ) ) ;
#47996=CARTESIAN_POINT ( 'NONE',  ( 33.44869771128058744, -277.5153814249955531, -298.7020541683110650 ) ) ;
#47997=CARTESIAN_POINT ( 'NONE',  ( 37.15087949335197237, -276.6471502468564267, -252.8641767520707901 ) ) ;
#47999=CARTESIAN_POINT ( 'NONE',  ( 35.02078894712537505, -275.2584812730623867, -260.7345828143970721 ) ) ;
#48000=CARTESIAN_POINT ( 'NONE',  ( -106.6505480030534869, -298.1835524515751672, -298.5801192096504906 ) ) ;
#48001=CARTESIAN_POINT ( 'NONE',  ( -41.39744745795693603, -284.0008302525749855, -195.6249535250933320 ) ) ;
#48002=CARTESIAN_POINT ( 'NONE',  ( -3.326869704139062911, -292.1557379576537414, -201.2905514753320517 ) ) ;
#48003=CARTESIAN_POINT ( 'NONE',  ( 32.66956441985474413, -273.2346496894775782, -244.4715517938489597 ) ) ;
#48004=CARTESIAN_POINT ( 'NONE',  ( 36.73160915207652977, -289.3788587385673736, -288.2932505926635258 ) ) ;
#48005=CARTESIAN_POINT ( 'NONE',  ( -12.14108662838064490, -291.3081128841067198, -201.4654860045028215 ) ) ;
#48007=CARTESIAN_POINT ( 'NONE',  ( -6.111030253669516910, -291.0292877846311512, -200.6099199626615359 ) ) ;
#48008=CARTESIAN_POINT ( 'NONE',  ( 31.82243232952892242, -292.9059329285202011, -246.7855275763157010 ) ) ;
#48010=CARTESIAN_POINT ( 'NONE',  ( 36.84888617535978739, -288.8759228471411689, -289.7840275117691249 ) ) ;
#48011=CARTESIAN_POINT ( 'NONE',  ( -83.45437583940538673, -279.7332126978419069, -213.6766918098673216 ) ) ;
#48012=CARTESIAN_POINT ( 'NONE',  ( -2.121727771319923850, -293.5172180888884554, -338.4863413428971626 ) ) ;
#48013=CARTESIAN_POINT ( 'NONE',  ( -108.9366198916925725, -285.5613768696180159, -242.1541868155274244 ) ) ;
#48015=CARTESIAN_POINT ( 'NONE',  ( 31.40100667542650115, -287.4395159495108487, -235.7174381439086801 ) ) ;
#48016=CARTESIAN_POINT ( 'NONE',  ( -4.813932744860490942, -282.9447479105849084, -335.7371979807689399 ) ) ;
#48017=CARTESIAN_POINT ( 'NONE',  ( 84.71888943659025983, 83.26956024130151945, -302.3639758324752620 ) ) ;
#48018=CARTESIAN_POINT ( 'NONE',  ( 201.7738562182570092, 295.5636489450776594, -54.00000000002855671 ) ) ;
#48019=CARTESIAN_POINT ( 'NONE',  ( -89.56232258695946769, -229.0018711643211873, -344.4782180464590624 ) ) ;
#48020=CARTESIAN_POINT ( 'NONE',  ( 19.30012945229858801, -275.4037526847995991, -316.6874952372622261 ) ) ;
#48021=CARTESIAN_POINT ( 'NONE',  ( 5.566627113730801213, -275.3762787172482831, -329.8636949792805240 ) ) ;
#48022=CARTESIAN_POINT ( 'NONE',  ( -36.89101025102353759, -297.5653089202770047, -193.4226924278395643 ) ) ;
#48023=CARTESIAN_POINT ( 'NONE',  ( -106.8704548483795662, -265.5134191007825279, -305.6964246945746595 ) ) ;
#48024=CARTESIAN_POINT ( 'NONE',  ( 36.11711466448170427, -273.9650309417401672, -248.7959255013256268 ) ) ;
#48025=CARTESIAN_POINT ( 'NONE',  ( -35.12482235915464202, -299.9406049207471483, -196.1251986654955601 ) ) ;
#48027=CARTESIAN_POINT ( 'NONE',  ( -37.61887856930841423, -298.9900076597199359, -193.5969115689300395 ) ) ;
#48028=CARTESIAN_POINT ( 'NONE',  ( 27.71007851628496255, -287.5916504390248747, -236.9891850880193545 ) ) ;
#48029=CARTESIAN_POINT ( 'NONE',  ( -110.6426745841473718, -297.0642769011980135, -293.4513091504965132 ) ) ;
#48030=CARTESIAN_POINT ( 'NONE',  ( -113.5416880409491398, -297.1787943969002868, -259.6314414746778994 ) ) ;
#48031=CARTESIAN_POINT ( 'NONE',  ( -68.51541026052402117, -295.6401757805547277, -336.3839378876151045 ) ) ;
#48033=CARTESIAN_POINT ( 'NONE',  ( 31.23566484959737721, -277.0572388499058434, -238.5118658668309308 ) ) ;
#48035=ORIENTED_EDGE ( 'NONE', *, *, #19214, .T. ) ;
#48036=CARTESIAN_POINT ( 'NONE',  ( -22.57184574353276929, -279.7438706481457302, -194.7994333121657462 ) ) ;
#48037=CARTESIAN_POINT ( 'NONE',  ( -29.67691765190060238, -277.8941220625322330, -343.2452823305832794 ) ) ;
#48038=CARTESIAN_POINT ( 'NONE',  ( -59.34981832276312730, -279.0933969597007831, -343.0908694280910822 ) ) ;
#48039=CARTESIAN_POINT ( 'NONE',  ( -72.10481659460799619, -275.5296269296171658, -337.2330637282659609 ) ) ;
#48040=CARTESIAN_POINT ( 'NONE',  ( -99.98842297843262372, -297.7223751282335229, -232.5893165343579199 ) ) ;
#48041=CARTESIAN_POINT ( 'NONE',  ( -47.89533903294519490, -293.7635801623702037, -343.2413491619556112 ) ) ;
#48043=CARTESIAN_POINT ( 'NONE',  ( -3.690190207552459523, -280.9766746888126363, -201.1577200415365780 ) ) ;
#48044=CARTESIAN_POINT ( 'NONE',  ( -96.40695242730352277, -279.3191981735195100, -227.4624469617730824 ) ) ;
#48045=CARTESIAN_POINT ( 'NONE',  ( -65.28262918174078777, -288.0945011380483720, -341.6393129022759467 ) ) ;
#48046=CARTESIAN_POINT ( 'NONE',  ( 17.68567777649750639, -300.7396324122937017, -195.1757337735481599 ) ) ;
#48048=CARTESIAN_POINT ( 'NONE',  ( -72.44530278041899862, -288.7266332883917812, -334.5509832891495421 ) ) ;
#48049=CARTESIAN_POINT ( 'NONE',  ( -19.26567184807625921, -278.5276300636957671, -198.5360193753688236 ) ) ;
#48050=CARTESIAN_POINT ( 'NONE',  ( -9.003806268212764863, -279.0049341340961746, -202.4469170409232675 ) ) ;
#48051=CARTESIAN_POINT ( 'NONE',  ( -18.39221623408244710, -280.8860927168760782, -342.4022665048565841 ) ) ;
#48052=CARTESIAN_POINT ( 'NONE',  ( -108.2281543000945447, -286.8711772596206515, -245.7075857765453009 ) ) ;
#48053=CARTESIAN_POINT ( 'NONE',  ( -91.60064415723140030, -280.4621314098903895, -220.9334182781018967 ) ) ;
#48056=CARTESIAN_POINT ( 'NONE',  ( -68.80792055221564851, -293.6387011374982308, -202.2672117711913984 ) ) ;
#48057=CARTESIAN_POINT ( 'NONE',  ( -59.39264490937714669, -275.5736814032318307, -343.0778962806397772 ) ) ;
#48058=CARTESIAN_POINT ( 'NONE',  ( -48.61538653169022695, -277.8507698712830916, -342.6399734491885738 ) ) ;
#48059=CARTESIAN_POINT ( 'NONE',  ( -84.92173646965555633, -285.7069368868990864, -328.5519124882036976 ) ) ;
#48061=CARTESIAN_POINT ( 'NONE',  ( -95.27101627565203046, -291.8067263863546259, -318.8941511515985212 ) ) ;
#48062=CARTESIAN_POINT ( 'NONE',  ( -34.10445267766981914, -293.0114124838975158, -345.3414397977035151 ) ) ;
#48063=CARTESIAN_POINT ( 'NONE',  ( -10.04174880431190964, -285.5967077281547404, -198.4791486451182152 ) ) ;
#48065=CARTESIAN_POINT ( 'NONE',  ( -11.29990959133293948, -273.0833919180785756, -201.5821161541705351 ) ) ;
#48066=CARTESIAN_POINT ( 'NONE',  ( 33.51891289664124685, -291.9800899656913202, -292.4889059963347790 ) ) ;
#48069=CARTESIAN_POINT ( 'NONE',  ( -108.8175379687289848, -289.3747428906872301, -243.4915026439281291 ) ) ;
#48070=CARTESIAN_POINT ( 'NONE',  ( -57.63370431021008500, -287.3860382586756259, -199.3524795963443523 ) ) ;
#48071=CARTESIAN_POINT ( 'NONE',  ( 27.84098234845882658, -285.2747797586742422, -231.2058855243546986 ) ) ;
#48072=CARTESIAN_POINT ( 'NONE',  ( -97.85069855169591335, -286.5564883452727827, -228.4576230561168302 ) ) ;
#48074=CARTESIAN_POINT ( 'NONE',  ( -49.45831668519996782, -286.6966947771290393, -198.1583483162472703 ) ) ;
#48075=CARTESIAN_POINT ( 'NONE',  ( -1.606573172722747245, -294.5033311058045342, -204.0180135460299198 ) ) ;
#48076=CARTESIAN_POINT ( 'NONE',  ( -8.458142772784642105, -274.7568828119530053, -340.1967224366917435 ) ) ;
#48077=CARTESIAN_POINT ( 'NONE',  ( 24.35325641475179737, -276.4980245334587039, -316.3988919163520563 ) ) ;
#48078=CARTESIAN_POINT ( 'NONE',  ( -3.935541531651221892, -290.5691221803448911, -202.5726450811971802 ) ) ;
#48079=CARTESIAN_POINT ( 'NONE',  ( -109.6061909089342947, -278.8899014647486183, -243.6206563244084577 ) ) ;
#48080=CARTESIAN_POINT ( 'NONE',  ( -112.0203564984756213, -298.5532047190371259, -268.7213695911513014 ) ) ;
#48083=CARTESIAN_POINT ( 'NONE',  ( -65.26517844446927086, -284.3643501987942841, -202.3251699399052939 ) ) ;
#48084=CARTESIAN_POINT ( 'NONE',  ( -103.2416664613760418, -277.1501380423098908, -236.0724180431797947 ) ) ;
#48085=CARTESIAN_POINT ( 'NONE',  ( 37.19810310196314163, -279.4396171916161506, -261.6093133841915233 ) ) ;
#48087=CARTESIAN_POINT ( 'NONE',  ( 24.77387833664412753, -273.4393883548008830, -226.0176265517116008 ) ) ;
#48088=CARTESIAN_POINT ( 'NONE',  ( -39.16861357176617275, -276.4242668820821223, -343.4402193438015161 ) ) ;
#48089=CARTESIAN_POINT ( 'NONE',  ( -12.75888253767304725, -296.2469795172567615, -339.8871329579883991 ) ) ;
#48090=CARTESIAN_POINT ( 'NONE',  ( 35.04052959382801191, -280.1497475699191000, -244.8586807805911576 ) ) ;
#48091=CARTESIAN_POINT ( 'NONE',  ( -10.39230126272301824, -295.6328916789736923, -338.4576549657351734 ) ) ;
#48092=CARTESIAN_POINT ( 'NONE',  ( -36.26448459679993164, -296.3541164526544094, -346.8734047659946214 ) ) ;
#48093=CARTESIAN_POINT ( 'NONE',  ( -68.04558847840438318, -297.4707818022457673, -204.1185230702592719 ) ) ;
#48094=CARTESIAN_POINT ( 'NONE',  ( -107.5927280713699190, -292.8950539665082715, -243.9496914794908946 ) ) ;
#48095=CARTESIAN_POINT ( 'NONE',  ( -43.66838422059648650, -286.1411151666180217, -193.5682139787643052 ) ) ;
#48096=CARTESIAN_POINT ( 'NONE',  ( 33.57407779989951280, -273.3488435027134074, -243.6916987981893783 ) ) ;
#48097=CARTESIAN_POINT ( 'NONE',  ( 34.04153349200878864, -287.7535908976397536, -299.3723852078082928 ) ) ;
#48098=CARTESIAN_POINT ( 'NONE',  ( -69.24873593890242773, -281.6101677387080713, -202.8793584270936492 ) ) ;
#48099=EDGE_CURVE ( 'NONE', #71727, #3540, #80024, .T. ) ;
#48100=CARTESIAN_POINT ( 'NONE',  ( 10.25913087916912758, -287.4355165199410749, -326.0839733444259991 ) ) ;
#48101=AXIS2_PLACEMENT_3D ( 'NONE', #69883, #70829, #91645 ) ;
#48102=CARTESIAN_POINT ( 'NONE',  ( -76.11297254768760467, -289.5343665862042144, -206.1000723414180982 ) ) ;
#48103=CARTESIAN_POINT ( 'NONE',  ( 206.7397234113112461, 289.2571863808457238, -82.84736978277094011 ) ) ;
#48104=CARTESIAN_POINT ( 'NONE',  ( 4.765946453601778821, -286.1453991372242740, -210.5921317269410622 ) ) ;
#48106=CARTESIAN_POINT ( 'NONE',  ( -5.542016770250216773, -283.5852327370769217, -340.2295683170670486 ) ) ;
#48107=CARTESIAN_POINT ( 'NONE',  ( -109.2492104208645429, -289.9535196269534367, -243.3372180496246813 ) ) ;
#48108=CARTESIAN_POINT ( 'NONE',  ( -28.33994573032229880, -281.7645389719714899, -194.6416201430762385 ) ) ;
#48109=CARTESIAN_POINT ( 'NONE',  ( 5.891699245674284491, -281.9402779481541188, -207.2408244923067855 ) ) ;
#48110=CARTESIAN_POINT ( 'NONE',  ( 17.96591689903805289, -280.7067189414089512, -222.6967033849904851 ) ) ;
#48111=CARTESIAN_POINT ( 'NONE',  ( -0.7690224333663998602, -276.5380006619288338, -204.8678694244426595 ) ) ;
#48112=CARTESIAN_POINT ( 'NONE',  ( -97.40743715241715961, -295.9064197607296478, -318.5598558583279214 ) ) ;
#48113=CARTESIAN_POINT ( 'NONE',  ( -102.5485085179513334, -289.0593478732129711, -233.9243277277530240 ) ) ;
#48114=CARTESIAN_POINT ( 'NONE',  ( -98.16367373487452141, -271.9161161942348031, -229.1874115693156568 ) ) ;
#48117=CARTESIAN_POINT ( 'NONE',  ( -100.8503879849079397, -286.9981649625802902, -231.4303869142295582 ) ) ;
#48118=CARTESIAN_POINT ( 'NONE',  ( 37.48537491343476091, -294.8435770192777454, -287.2252398383371315 ) ) ;
#48119=CARTESIAN_POINT ( 'NONE',  ( 18.57768135893347150, -282.8716615639164615, -317.4646838326616489 ) ) ;
#48120=CARTESIAN_POINT ( 'NONE',  ( 0.9193240794713762876, -275.6137808110120204, -336.9714951117172177 ) ) ;
#48121=CARTESIAN_POINT ( 'NONE',  ( -114.1490865168415496, -291.1568109996039766, -274.0945055092949474 ) ) ;
#48122=CARTESIAN_POINT ( 'NONE',  ( -60.11569579609300007, -283.8997746002893905, -198.0454504107334230 ) ) ;
#48123=CARTESIAN_POINT ( 'NONE',  ( -69.61816762772461686, -291.9720920344217916, -200.4613457950580937 ) ) ;
#48124=CARTESIAN_POINT ( 'NONE',  ( 33.40799360663910988, -287.6463735253017830, -252.2394594944182415 ) ) ;
#48127=CARTESIAN_POINT ( 'NONE',  ( 201.2023760237154022, 289.8772717810621771, -82.34854583857284638 ) ) ;
#48128=CARTESIAN_POINT ( 'NONE',  ( -31.66834704498080910, -284.5019116313486052, -346.4697382252610964 ) ) ;
#48129=CARTESIAN_POINT ( 'NONE',  ( -37.37352853689063181, -280.5523547857346784, -345.3611179825600175 ) ) ;
#48131=CARTESIAN_POINT ( 'NONE',  ( 34.37044507695362228, -280.2718136640810940, -255.0830286507073197 ) ) ;
#48132=CARTESIAN_POINT ( 'NONE',  ( 38.71419002419975186, -275.3717312788068625, -282.5802417195464500 ) ) ;
#48133=CARTESIAN_POINT ( 'NONE',  ( -65.52973139678472592, -281.6828876221191535, -201.0396687706584942 ) ) ;
#48134=CARTESIAN_POINT ( 'NONE',  ( 86.48509054211875480, 81.40261763058097699, -300.6191915867298121 ) ) ;
#48135=CARTESIAN_POINT ( 'NONE',  ( -2.641384495198680238, -279.0766083356290892, -202.2693806509963395 ) ) ;
#48136=CARTESIAN_POINT ( 'NONE',  ( -80.23426965169983305, -283.4886673868447247, -209.2069716719045687 ) ) ;
#48137=CARTESIAN_POINT ( 'NONE',  ( -112.3254095316165575, -274.5550457451084299, -259.1513055606759508 ) ) ;
#48139=CARTESIAN_POINT ( 'NONE',  ( 34.77367263360802241, -293.8889931390622792, -258.5627964123414699 ) ) ;
#48141=CARTESIAN_POINT ( 'NONE',  ( -69.21643514041636536, -290.3086991821817833, -204.1260422614612651 ) ) ;
#48142=CARTESIAN_POINT ( 'NONE',  ( 16.88923124050585400, -276.9560013031302788, -324.9544579712895711 ) ) ;
#48143=CARTESIAN_POINT ( 'NONE',  ( -35.39032682862060142, -274.0772884858102429, -197.3746985426482752 ) ) ;
#48144=CARTESIAN_POINT ( 'NONE',  ( -108.8732912634602314, -271.8258429508988456, -242.5613660887286187 ) ) ;
#48146=CARTESIAN_POINT ( 'NONE',  ( 31.39124254195288444, -273.1576487003497959, -240.2202605137360081 ) ) ;
#48148=CARTESIAN_POINT ( 'NONE',  ( 35.33738724059130476, -282.5008974009485883, -260.3938012047546522 ) ) ;
#48149=CARTESIAN_POINT ( 'NONE',  ( 20.84865420022137883, -283.9789812043584902, -319.2268184223113963 ) ) ;
#48150=CARTESIAN_POINT ( 'NONE',  ( -110.4210618144994811, -283.8576144872841951, -273.6344385098506109 ) ) ;
#48151=CARTESIAN_POINT ( 'NONE',  ( -27.15986309337434790, -272.5834449228148628, -197.2154022288762008 ) ) ;
#48152=CARTESIAN_POINT ( 'NONE',  ( -2.591510683314547148, -282.3771793671254500, -204.7472373271185404 ) ) ;
#48153=CARTESIAN_POINT ( 'NONE',  ( 36.07072427727253228, -273.9407200308869506, -263.3740828805771343 ) ) ;
#48155=CARTESIAN_POINT ( 'NONE',  ( 30.45546947606247556, -276.2580272155894363, -242.3393587185985041 ) ) ;
#48157=CARTESIAN_POINT ( 'NONE',  ( -35.35048106932609358, -280.8793458563240506, -193.5352891781130609 ) ) ;
#48161=CARTESIAN_POINT ( 'NONE',  ( -89.06065693698418784, -287.1950952844992457, -214.9231892402815731 ) ) ;
#48162=CARTESIAN_POINT ( 'NONE',  ( -90.53164746971077648, -295.0266919885551715, -320.6678543587751733 ) ) ;
#48164=CARTESIAN_POINT ( 'NONE',  ( -112.1654381582483069, -289.6778751024993426, -288.1578626059623502 ) ) ;
#48165=CARTESIAN_POINT ( 'NONE',  ( 24.39149250408241087, -285.2322303745413024, -229.4395364344854329 ) ) ;
#48166=CARTESIAN_POINT ( 'NONE',  ( 29.35156276043435497, -285.7102677632536256, -239.2583270995723410 ) ) ;
#48167=CARTESIAN_POINT ( 'NONE',  ( -91.48540141591061570, -289.5078895091708091, -219.8801859189374852 ) ) ;
#48169=CARTESIAN_POINT ( 'NONE',  ( -94.58510355949549364, -285.1113264748915412, -316.3193605643512569 ) ) ;
#48170=CARTESIAN_POINT ( 'NONE',  ( -26.09567069839383180, -274.9087881577153780, -344.5131743840228182 ) ) ;
#48171=CARTESIAN_POINT ( 'NONE',  ( 24.90351194010699132, -285.3640387415452437, -226.3843873973165444 ) ) ;
#48172=CARTESIAN_POINT ( 'NONE',  ( -103.5016762719473462, -299.0222371892259616, -234.9258414638996726 ) ) ;
#48173=CARTESIAN_POINT ( 'NONE',  ( 4.188483759107254123, -284.6098817907607668, -207.6471174207159152 ) ) ;
#48174=CARTESIAN_POINT ( 'NONE',  ( -3.049495471550309311, -281.4581639829564210, -205.6363620462592792 ) ) ;
#48175=CARTESIAN_POINT ( 'NONE',  ( -3.854061793760648946, -290.6116789360389134, -337.6703220621185437 ) ) ;
#48178=CARTESIAN_POINT ( 'NONE',  ( -65.05220623504222033, -297.3315034624819191, -340.6704632836123778 ) ) ;
#48179=CARTESIAN_POINT ( 'NONE',  ( -103.9198863114396119, -277.0104159929051093, -235.7178019441233516 ) ) ;
#48180=CARTESIAN_POINT ( 'NONE',  ( 19.30354945160366142, -292.0415279096809513, -218.4431584635558465 ) ) ;
#48181=CARTESIAN_POINT ( 'NONE',  ( -95.41545011542045529, -294.3168545863970849, -315.9009904023843092 ) ) ;
#48182=CARTESIAN_POINT ( 'NONE',  ( 18.86073536142054508, -280.9053923955477785, -317.7360035651342969 ) ) ;
#48183=CARTESIAN_POINT ( 'NONE',  ( -59.88897828414093993, -271.8377124552929445, -199.3639816523339903 ) ) ;
#48184=CARTESIAN_POINT ( 'NONE',  ( 28.84592326470875889, -295.2981185180726698, -302.4228937726682602 ) ) ;
#48185=CARTESIAN_POINT ( 'NONE',  ( 21.27581636871892101, -295.4090924074130839, -223.5744983911110353 ) ) ;
#48186=CARTESIAN_POINT ( 'NONE',  ( -111.9315635258766548, -294.8289132191052886, -286.4564599686050883 ) ) ;
#48187=CARTESIAN_POINT ( 'NONE',  ( 32.47651884501699016, -292.1806182556719591, -300.4837451469400662 ) ) ;
#48188=CARTESIAN_POINT ( 'NONE',  ( -89.06240403470538070, -291.2223359890217012, -322.7094102557475708 ) ) ;
#48190=CARTESIAN_POINT ( 'NONE',  ( -28.09605347149809518, -292.9752033197778474, -197.7353328131947876 ) ) ;
#48192=CARTESIAN_POINT ( 'NONE',  ( -109.4863796075772910, -291.4287114631408144, -296.2700622463460718 ) ) ;
#48193=CARTESIAN_POINT ( 'NONE',  ( 12.57203154460730765, -280.3810623515549878, -326.8843052278369896 ) ) ;
#48194=CARTESIAN_POINT ( 'NONE',  ( -28.10634817360825011, -292.1725000703404476, -197.8969160183965528 ) ) ;
#48195=CARTESIAN_POINT ( 'NONE',  ( -6.230367260804436036, -280.4497173260231762, -199.9118759752091705 ) ) ;
#48196=CARTESIAN_POINT ( 'NONE',  ( -104.4006824616695042, -283.7270248147945608, -308.2690538005964527 ) ) ;
#48197=CARTESIAN_POINT ( 'NONE',  ( 24.24457226759903605, -286.1298346627839351, -312.8943929153469412 ) ) ;
#48198=CARTESIAN_POINT ( 'NONE',  ( -45.80340010422668229, -281.2999921081806747, -344.1643498713454505 ) ) ;
#48199=LINE ( 'NONE', #56272, #57865 ) ;
#48200=CARTESIAN_POINT ( 'NONE',  ( -70.91197008725632145, -278.0971406944752857, -201.8356137489730031 ) ) ;
#48201=CARTESIAN_POINT ( 'NONE',  ( -35.14326549877506523, -284.9994502276404660, -193.6886549248184224 ) ) ;
#48202=CARTESIAN_POINT ( 'NONE',  ( 31.33745725645997737, -295.5112275111496842, -297.5124002757800667 ) ) ;
#48203=CARTESIAN_POINT ( 'NONE',  ( 18.48520459717543574, -277.6944423838507419, -322.5335532492172774 ) ) ;
#48204=CARTESIAN_POINT ( 'NONE',  ( -29.71543538952376906, -276.6197943412473137, -343.0338504192867504 ) ) ;
#48205=CARTESIAN_POINT ( 'NONE',  ( -113.1723885649860790, -290.8860182774737950, -256.9929956124397563 ) ) ;
#48206=CARTESIAN_POINT ( 'NONE',  ( 18.69876228800809415, -280.3340898087510595, -321.1207778022061348 ) ) ;
#48207=CARTESIAN_POINT ( 'NONE',  ( 35.94337457124368740, -292.6163125183845750, -270.7731708454860495 ) ) ;
#48208=CARTESIAN_POINT ( 'NONE',  ( -109.3037970399574021, -294.2793639761447935, -291.5360056562745967 ) ) ;
#48211=CARTESIAN_POINT ( 'NONE',  ( -28.89508416255553769, -294.4499753546238594, -342.9838155983697447 ) ) ;
#48212=DIRECTION ( 'NONE',  ( 1.000000000000000000, 0.000000000000000000, 0.000000000000000000 ) ) ;
#48213=CARTESIAN_POINT ( 'NONE',  ( -109.1418805571601069, -282.0523547857346784, -270.3284710469131937 ) ) ;
#48214=CARTESIAN_POINT ( 'NONE',  ( -91.46112644410375481, -296.3630665602345857, -215.9193334063130862 ) ) ;
#48215=CARTESIAN_POINT ( 'NONE',  ( 38.38447587388164806, -279.7224820264187883, -272.7801562233553341 ) ) ;
#48218=CARTESIAN_POINT ( 'NONE',  ( -64.38862046288612362, -287.0216211162978652, -198.7805505694091153 ) ) ;
#48219=CARTESIAN_POINT ( 'NONE',  ( 21.99282024748162456, -286.7900700911326908, -227.7504317409685370 ) ) ;
#48220=CARTESIAN_POINT ( 'NONE',  ( -59.38411559195876777, -278.8629099092265164, -340.6806719609382412 ) ) ;
#48221=CARTESIAN_POINT ( 'NONE',  ( -106.4949680734156487, -294.2041406121150544, -298.4622270833087896 ) ) ;
#48222=CARTESIAN_POINT ( 'NONE',  ( -80.73096090367614863, -297.4101122009274718, -330.3223226113856867 ) ) ;
#48223=CARTESIAN_POINT ( 'NONE',  ( -107.5007011856816774, -277.0610164495790855, -292.0916920042543552 ) ) ;
#48226=CARTESIAN_POINT ( 'NONE',  ( -103.8293999450873883, -296.7250128119463852, -231.4600736546301789 ) ) ;
#48227=CARTESIAN_POINT ( 'NONE',  ( -111.4080644413768795, -292.5686752247817708, -262.9120996640185695 ) ) ;
#48228=CARTESIAN_POINT ( 'NONE',  ( 37.82059482285082197, -295.3116620276945241, -282.9730546295761542 ) ) ;
#48229=CARTESIAN_POINT ( 'NONE',  ( 201.2258855950020120, 292.9574286262273404, -53.99999999998392042 ) ) ;
#48230=CARTESIAN_POINT ( 'NONE',  ( -61.28057334557731650, -290.0228310720435161, -339.4322625883503974 ) ) ;
#48232=CARTESIAN_POINT ( 'NONE',  ( 39.04270912039385166, -280.7130715193023320, -278.5055142916631894 ) ) ;
#48233=CARTESIAN_POINT ( 'NONE',  ( -105.8631005652257500, -296.7521921598509493, -305.3801170956911619 ) ) ;
#48234=CARTESIAN_POINT ( 'NONE',  ( -104.0793199474377673, -288.2204817048622658, -306.2274751834333415 ) ) ;
#48235=AXIS2_PLACEMENT_3D ( 'NONE', #55562, #4886, #83954 ) ;
#48236=CARTESIAN_POINT ( 'NONE',  ( 76.34370912324891378, -299.7723574772524557, -193.3759528850984850 ) ) ;
#48239=DIRECTION ( 'NONE',  ( 0.000000000000000000, 0.000000000000000000, 1.000000000000000000 ) ) ;
#48240=CARTESIAN_POINT ( 'NONE',  ( -2.103535665248870146, -290.1142860229408029, -338.0440517228934709 ) ) ;
#48241=CARTESIAN_POINT ( 'NONE',  ( 44.71564893372296723, -284.0519495502702512, -270.3284710469131937 ) ) ;
#48243=CARTESIAN_POINT ( 'NONE',  ( 37.58007017541937955, -280.6831690714219008, -252.9815412302551181 ) ) ;
#48244=CARTESIAN_POINT ( 'NONE',  ( -112.1504076022523151, -286.5087614331251302, -273.7458378903837115 ) ) ;
#48245=CARTESIAN_POINT ( 'NONE',  ( 37.14931278864178665, -285.9117211328272674, -253.2825489496468094 ) ) ;
#48246=CARTESIAN_POINT ( 'NONE',  ( 34.63013171584941574, -273.2854874025736649, -249.6797832033184648 ) ) ;
#48247=CARTESIAN_POINT ( 'NONE',  ( -77.35853366648174756, -275.4309988540003360, -207.5919597100882186 ) ) ;
#48248=CARTESIAN_POINT ( 'NONE',  ( -90.83444329595218392, -289.3656453919955425, -218.5939408731165656 ) ) ;
#48249=CARTESIAN_POINT ( 'NONE',  ( -108.5673249219375407, -280.0792343271966729, -296.3449803599485222 ) ) ;
#48250=CARTESIAN_POINT ( 'NONE',  ( -62.30894776949511282, -279.7182842829084848, -201.7101182751092097 ) ) ;
#48251=CARTESIAN_POINT ( 'NONE',  ( -16.88525478471229491, -279.6720178844207112, -200.1797350393848944 ) ) ;
#48252=CARTESIAN_POINT ( 'NONE',  ( -31.46019730038518247, -278.0593344818556147, -346.8785573851295680 ) ) ;
#48253=CARTESIAN_POINT ( 'NONE',  ( 37.59942885551402725, -280.1467957857979059, -254.4289681991214138 ) ) ;
#48254=CARTESIAN_POINT ( 'NONE',  ( 137.1361844366198284, 179.7607878149970873, -239.0752527614820906 ) ) ;
#48255=CARTESIAN_POINT ( 'NONE',  ( 17.91188411107352962, -275.7607703711248632, -216.9944729222064552 ) ) ;
#48257=CARTESIAN_POINT ( 'NONE',  ( -113.1758016124685469, -274.1792792852132266, -261.8819196752850189 ) ) ;
#48258=CARTESIAN_POINT ( 'NONE',  ( -95.95921662488163406, -292.4090924074130839, -317.1477375740089997 ) ) ;
#48259=ORIENTED_EDGE ( 'NONE', *, *, #20584, .F. ) ;
#48261=CARTESIAN_POINT ( 'NONE',  ( 33.68464352486044078, -288.3926430302678341, -252.1587781654427545 ) ) ;
#48262=CARTESIAN_POINT ( 'NONE',  ( 38.08754324716364437, -289.4340977047092451, -279.9724771504866112 ) ) ;
#48263=CARTESIAN_POINT ( 'NONE',  ( -71.22736778932592472, -288.8604619849172082, -335.1491306327570214 ) ) ;
#48264=CARTESIAN_POINT ( 'NONE',  ( -89.83966968000169118, -284.8427110194635361, -214.0437511867768308 ) ) ;
#48265=CARTESIAN_POINT ( 'NONE',  ( -55.04033302849770593, -170.0623274831404501, -364.4220463826554237 ) ) ;
#48266=CARTESIAN_POINT ( 'NONE',  ( -33.47446041278221429, -281.4025652945214802, -344.0724367632854523 ) ) ;
#48267=CARTESIAN_POINT ( 'NONE',  ( 0.7830223900123518543, -288.4264218532675841, -206.6037034371304628 ) ) ;
#48268=CARTESIAN_POINT ( 'NONE',  ( 5.984242604995782422, -280.9322072682146541, -329.9729493334255039 ) ) ;
#48269=CARTESIAN_POINT ( 'NONE',  ( -46.53463803143360167, -281.2483632428370015, -197.3937359102122855 ) ) ;
#48270=CARTESIAN_POINT ( 'NONE',  ( -59.20744856401751832, -277.8353006702819243, -340.0739395211526244 ) ) ;
#48271=CARTESIAN_POINT ( 'NONE',  ( -87.13802472664364984, -288.5225688464320797, -328.6402068824518210 ) ) ;
#48272=CARTESIAN_POINT ( 'NONE',  ( -111.5679106737709674, -285.6065000147708588, -250.2957787312075197 ) ) ;
#48273=CARTESIAN_POINT ( 'NONE',  ( -97.12061319322400266, -284.3941279144026453, -318.8174311157850411 ) ) ;
#48274=CARTESIAN_POINT ( 'NONE',  ( 35.56602825606886853, -281.7672363353926244, -274.0303340226344631 ) ) ;
#48277=CARTESIAN_POINT ( 'NONE',  ( -98.85336085966375208, -291.8164170333934635, -314.6170461761369097 ) ) ;
#48278=CARTESIAN_POINT ( 'NONE',  ( -2.266904459064136734, -291.1912931058530489, -202.3533679012895732 ) ) ;
#48279=CARTESIAN_POINT ( 'NONE',  ( 15.62522702115081152, -273.8830356304416114, -219.7118805459503221 ) ) ;
#48280=CARTESIAN_POINT ( 'NONE',  ( -68.19290821783590673, -294.7954055040969479, -340.7991456826188141 ) ) ;
#48281=CARTESIAN_POINT ( 'NONE',  ( -57.82930486894797184, -290.2627198948393357, -199.5195675322050874 ) ) ;
#48282=CARTESIAN_POINT ( 'NONE',  ( -87.18875795470485457, -293.9981015954780332, -325.0716730659176505 ) ) ;
#48283=CARTESIAN_POINT ( 'NONE',  ( -106.4010151430424429, -291.4279441581856531, -295.2195474187745390 ) ) ;
#48285=CARTESIAN_POINT ( 'NONE',  ( -107.9732148254756510, -292.2236681064712229, -295.7377400441716304 ) ) ;
#48286=CARTESIAN_POINT ( 'NONE',  ( -36.37571562165233985, -290.0640810556073461, -195.1879316464278702 ) ) ;
#48287=CARTESIAN_POINT ( 'NONE',  ( 34.13697829171586307, -295.8473533208329513, -293.2405296360474836 ) ) ;
#48288=CARTESIAN_POINT ( 'NONE',  ( -85.89106717455422313, -286.3015191168598790, -215.4629765413057214 ) ) ;
#48289=CARTESIAN_POINT ( 'NONE',  ( 7.825334897150399094, -296.4369795928970461, -330.4441219903541196 ) ) ;
#48290=CARTESIAN_POINT ( 'NONE',  ( 16.88800983094458275, -276.7992430895737357, -217.9646831585044140 ) ) ;
#48292=CARTESIAN_POINT ( 'NONE',  ( -80.52580401830833523, -296.6804488125075068, -206.7417257793347289 ) ) ;
#48293=CARTESIAN_POINT ( 'NONE',  ( -18.78421973913642162, -275.0497598008045657, -342.0102207865367632 ) ) ;
#48294=CARTESIAN_POINT ( 'NONE',  ( -30.09839855958027144, -278.2242163915004767, -196.2230040988926589 ) ) ;
#48295=CARTESIAN_POINT ( 'NONE',  ( -64.73113572071081023, -274.8914451269762935, -202.2524143782383703 ) ) ;
#48296=CARTESIAN_POINT ( 'NONE',  ( 21.40953634539815553, -273.4647390110447986, -221.5052226612841935 ) ) ;
#48297=CARTESIAN_POINT ( 'NONE',  ( -47.85945287511258073, -296.6136657269190664, -343.2465373170531961 ) ) ;
#48299=CARTESIAN_POINT ( 'NONE',  ( -110.2592475881748726, -297.2686014344033651, -276.9242794681202895 ) ) ;
#48302=CARTESIAN_POINT ( 'NONE',  ( -34.74920894124682036, -287.0398363969529782, -345.6717134848606179 ) ) ;
#48303=CARTESIAN_POINT ( 'NONE',  ( -76.56243908317212288, -273.3445010671472915, -208.7921839304540583 ) ) ;
#48304=CARTESIAN_POINT ( 'NONE',  ( -12.70370912436400346, -286.3638245121680370, -197.4092886751276410 ) ) ;
#48306=CARTESIAN_POINT ( 'NONE',  ( -3.073958341812169426, -288.2786149031339846, -339.3066218145507946 ) ) ;
#48307=CARTESIAN_POINT ( 'NONE',  ( -110.3682943135602414, -298.2937635201168405, -289.0013984510330829 ) ) ;
#48308=CARTESIAN_POINT ( 'NONE',  ( 27.36546434194725919, -292.0550941575467050, -307.9511604220298295 ) ) ;
#48309=CARTESIAN_POINT ( 'NONE',  ( 26.58186677002952791, -281.3117356188814142, -312.9983835544960016 ) ) ;
#48310=CARTESIAN_POINT ( 'NONE',  ( -69.91165696735023971, -292.9809262143061801, -337.9199732462171255 ) ) ;
#48311=CARTESIAN_POINT ( 'NONE',  ( -40.23143059711612324, -278.0158033824083077, -195.3666499803061640 ) ) ;
#48313=CARTESIAN_POINT ( 'NONE',  ( -13.17151362372341161, -287.5259493857911934, -339.6643111905694923 ) ) ;
#48314=CARTESIAN_POINT ( 'NONE',  ( 145.2857639756989272, -299.5541904835127980, -195.3611179825600175 ) ) ;
#48315=CARTESIAN_POINT ( 'NONE',  ( -104.6512700280956096, -288.1156943258516776, -303.4431742292746321 ) ) ;
#48316=CARTESIAN_POINT ( 'NONE',  ( -109.8151229117183050, -274.2503445683700534, -256.7344692846174894 ) ) ;
#48317=CARTESIAN_POINT ( 'NONE',  ( -30.25136146452663510, -284.3893788874253801, -346.4422154389332604 ) ) ;
#48318=CARTESIAN_POINT ( 'NONE',  ( -40.34881800459285728, -296.0347712644656895, -195.0149243524149085 ) ) ;
#48319=CARTESIAN_POINT ( 'NONE',  ( 32.73458966462342801, -281.2815865231557950, -249.9084015642242775 ) ) ;
#48320=CARTESIAN_POINT ( 'NONE',  ( -112.2748472428251034, -296.9404662471065421, -252.6404106598941155 ) ) ;
#48321=CARTESIAN_POINT ( 'NONE',  ( -35.39276809505724231, -275.5023302713062776, -196.7850927431614707 ) ) ;
#48322=CARTESIAN_POINT ( 'NONE',  ( 37.64001326412503801, -283.5106729013216409, -267.1177837441419456 ) ) ;
#48323=CARTESIAN_POINT ( 'NONE',  ( -93.14015919119425746, -272.1461418700350237, -222.7943157374531324 ) ) ;
#48326=CARTESIAN_POINT ( 'NONE',  ( -73.18549626151961718, -287.5544330567582278, -204.8708652353481909 ) ) ;
#48328=CARTESIAN_POINT ( 'NONE',  ( -2.602324593224659921, -277.9809262143061233, -198.2974183793908196 ) ) ;
#48329=CARTESIAN_POINT ( 'NONE',  ( -113.5555853299319296, -277.8769297596418255, -260.1791036389054739 ) ) ;
#48331=CARTESIAN_POINT ( 'NONE',  ( -108.0636303958906552, -288.5882183118450257, -298.7309786267562117 ) ) ;
#48332=CARTESIAN_POINT ( 'NONE',  ( -40.24245257090158390, -284.6093989717445538, -343.9973413310283945 ) ) ;
#48333=CARTESIAN_POINT ( 'NONE',  ( 18.93149402914985302, -277.8237901899742042, -318.1080344928448653 ) ) ;
#48334=CARTESIAN_POINT ( 'NONE',  ( -102.4067645159229443, -285.4497173072661553, -310.4253624932176763 ) ) ;
#48335=CARTESIAN_POINT ( 'NONE',  ( -92.86953636848627980, -282.6667304108290750, -318.3780606137623295 ) ) ;
#48336=CARTESIAN_POINT ( 'NONE',  ( 28.19444638708343120, -283.0669582107580027, -233.8917589790296745 ) ) ;
#48337=CARTESIAN_POINT ( 'NONE',  ( -2.559442880076310711, -274.6660035731552512, -201.6500210935546136 ) ) ;
#48338=CARTESIAN_POINT ( 'NONE',  ( -103.6068740789867348, -277.8734136366252869, -309.6820917713292829 ) ) ;
#48339=CARTESIAN_POINT ( 'NONE',  ( -61.45698932821379401, -297.2878551452225793, -340.8413559345464705 ) ) ;
#48340=DIRECTION ( 'NONE',  ( 0.000000000000000000, 0.000000000000000000, -1.000000000000000000 ) ) ;
#48342=CARTESIAN_POINT ( 'NONE',  ( -85.62663953305602149, -293.8517246473459750, -328.7466479061922087 ) ) ;
#48343=CARTESIAN_POINT ( 'NONE',  ( 33.95193598306571658, -275.2711147623555235, -286.3931504640509615 ) ) ;
#48344=CARTESIAN_POINT ( 'NONE',  ( -29.11472206127396589, -299.2325517387172908, -193.6687589893388974 ) ) ;
#48345=CARTESIAN_POINT ( 'NONE',  ( -37.30253330699734704, -287.8127541948342696, -196.3351800257841830 ) ) ;
#48346=CARTESIAN_POINT ( 'NONE',  ( 19.03066992430094473, -295.7784688558535322, -321.8663426198303341 ) ) ;
#48347=CARTESIAN_POINT ( 'NONE',  ( 36.69483933173619761, -294.5092082844912511, -250.6484148318101006 ) ) ;
#48348=CARTESIAN_POINT ( 'NONE',  ( -93.05468292082453274, -293.2499372506653685, -220.3810392619222682 ) ) ;
#48349=CARTESIAN_POINT ( 'NONE',  ( -57.58528846773011622, -277.7900246710119632, -198.3178979343840922 ) ) ;
#48350=CARTESIAN_POINT ( 'NONE',  ( -60.19858852931782423, -281.6738427201626678, -199.4627235524875744 ) ) ;
#48351=CARTESIAN_POINT ( 'NONE',  ( -61.50323121599836185, -293.4481658126289290, -340.8255182577509004 ) ) ;
#48352=CARTESIAN_POINT ( 'NONE',  ( -92.51552991585175789, -285.6920635472461640, -322.3046338264631459 ) ) ;
#48353=CARTESIAN_POINT ( 'NONE',  ( -110.3006262632761008, -283.5730573429611354, -262.7041560976790606 ) ) ;
#48354=CARTESIAN_POINT ( 'NONE',  ( -69.03337401324819211, -197.1869525245530497, -359.5623982929876092 ) ) ;
#48356=CARTESIAN_POINT ( 'NONE',  ( -83.65800552672159540, -285.0631796683132393, -213.8429002867146949 ) ) ;
#48357=VERTEX_POINT ( 'NONE', #70705 ) ;
#48358=CARTESIAN_POINT ( 'NONE',  ( 37.84522866867033741, -282.8215958024190400, -285.4746301119304235 ) ) ;
#48359=CARTESIAN_POINT ( 'NONE',  ( -40.78018372585002993, -274.3411336451096645, -197.3712610901739595 ) ) ;
#48360=CARTESIAN_POINT ( 'NONE',  ( -10.12063317540506624, -285.1945294551290999, -198.7013773986871001 ) ) ;
#48361=CARTESIAN_POINT ( 'NONE',  ( 38.56022927156001145, -282.3451071180677445, -258.5398940096742422 ) ) ;
#48362=CARTESIAN_POINT ( 'NONE',  ( -88.73077615254480577, -279.2783275606940379, -326.7691902467350360 ) ) ;
#48363=CARTESIAN_POINT ( 'NONE',  ( -50.92977659393751821, -280.5342955611226330, -194.6730940669284848 ) ) ;
#48365=CARTESIAN_POINT ( 'NONE',  ( 17.40634833298269157, -272.4094976428775681, -226.7417163044926838 ) ) ;
#48366=CARTESIAN_POINT ( 'NONE',  ( -112.8250949930600342, -274.3352372842284694, -284.1850902867908530 ) ) ;
#48368=CARTESIAN_POINT ( 'NONE',  ( -32.59967766544144041, -276.1122001132225705, -195.6653361609325827 ) ) ;
#48369=CARTESIAN_POINT ( 'NONE',  ( 24.68374711691411250, -22.60613715962459835, -344.8050946662477259 ) ) ;
#48370=CIRCLE ( 'NONE', #72595, 1.000000000000000888 ) ;
#48371=CARTESIAN_POINT ( 'NONE',  ( -13.76600370310567989, -278.3795911341124452, -199.4825077167134282 ) ) ;
#48372=CARTESIAN_POINT ( 'NONE',  ( -25.20566085914393639, -293.9649894280912008, -195.3498484120852083 ) ) ;
#48373=CARTESIAN_POINT ( 'NONE',  ( -63.61336347081373077, -294.7523016461514089, -338.6327307080335913 ) ) ;
#48374=CARTESIAN_POINT ( 'NONE',  ( -86.46891560568977297, -290.8988238997511644, -211.0800931791311541 ) ) ;
#48376=CARTESIAN_POINT ( 'NONE',  ( -102.6216885265388470, -294.6043399248806622, -310.0742065885632996 ) ) ;
#48377=CARTESIAN_POINT ( 'NONE',  ( 23.39685592856236696, -286.5298021907969428, -312.3031679155489542 ) ) ;
#48378=CARTESIAN_POINT ( 'NONE',  ( 36.52187393452328479, -295.3099115456131472, -262.4470789572811782 ) ) ;
#48379=CARTESIAN_POINT ( 'NONE',  ( -103.9393927611244379, -286.2856263280274334, -239.1600271303572640 ) ) ;
#48380=CARTESIAN_POINT ( 'NONE',  ( -39.21799212274207491, -292.9704245363171253, -193.6063496476391208 ) ) ;
#48381=CARTESIAN_POINT ( 'NONE',  ( -21.36865974107884014, -283.3342165910232211, -341.7072876758564917 ) ) ;
#48382=CARTESIAN_POINT ( 'NONE',  ( -76.89044581166889714, -294.3639536327408450, -336.0269928067512524 ) ) ;
#48383=CARTESIAN_POINT ( 'NONE',  ( -93.46783919006307428, -290.6371201916478526, -322.9165015005222017 ) ) ;
#48384=CARTESIAN_POINT ( 'NONE',  ( -105.0988082359836682, -290.5728660934659047, -306.8097284351090934 ) ) ;
#48385=CARTESIAN_POINT ( 'NONE',  ( 34.28456961682574189, -287.9056257663229985, -284.5210461893441902 ) ) ;
#48388=CARTESIAN_POINT ( 'NONE',  ( -106.6527944323064929, -298.8107939000017268, -239.6326587553027991 ) ) ;
#48389=CARTESIAN_POINT ( 'NONE',  ( -112.6507146381146924, -295.4067209459291234, -256.8759184266080524 ) ) ;
#48390=CARTESIAN_POINT ( 'NONE',  ( 17.24617079671854114, -279.9146824177398116, -221.5392704513667468 ) ) ;
#48392=CARTESIAN_POINT ( 'NONE',  ( 7.204470190248506434, -274.1485267188602393, -207.5648335849591604 ) ) ;
#48393=CARTESIAN_POINT ( 'NONE',  ( -111.0674747947812477, -295.0537537471150813, -268.6981155592530399 ) ) ;
#48394=CARTESIAN_POINT ( 'NONE',  ( -32.31362477967866909, -278.8486366233668150, -344.4766572952412957 ) ) ;
#48395=CARTESIAN_POINT ( 'NONE',  ( -43.56240282120956664, -272.1124542684461858, -196.3354438154922263 ) ) ;
#48396=CARTESIAN_POINT ( 'NONE',  ( -105.3239414312393052, -297.3885957285963286, -298.0296085683576166 ) ) ;
#48397=CARTESIAN_POINT ( 'NONE',  ( -109.0844819342029837, -297.8306052815145222, -255.2275716800408532 ) ) ;
#48399=CARTESIAN_POINT ( 'NONE',  ( -61.32029111936589061, -296.9584460591776178, -342.7451568002657041 ) ) ;
#48400=CARTESIAN_POINT ( 'NONE',  ( -95.64702959962350803, -271.2274239832901230, -222.6032128009957205 ) ) ;
#48401=CARTESIAN_POINT ( 'NONE',  ( -12.23297577692504490, -293.0389183995652047, -201.6526366028926134 ) ) ;
#48402=CARTESIAN_POINT ( 'NONE',  ( -109.2828030577999101, -289.3295433326570105, -254.8739417330797039 ) ) ;
#48404=CARTESIAN_POINT ( 'NONE',  ( 37.84687850303124890, -276.2494818356835253, -286.7384708335228538 ) ) ;
#48405=CARTESIAN_POINT ( 'NONE',  ( -108.4985990204608015, -297.1016445856391215, -253.9665082921558792 ) ) ;
#48406=CARTESIAN_POINT ( 'NONE',  ( -39.56455599133202838, -282.0042896937175669, -195.0259346131890652 ) ) ;
#48407=CARTESIAN_POINT ( 'NONE',  ( 36.51337515722941873, -279.9847435268589493, -250.3432676603068501 ) ) ;
#48408=CARTESIAN_POINT ( 'NONE',  ( -62.38065179035082508, -276.7179619073056642, -343.1247379986887154 ) ) ;
#48409=CARTESIAN_POINT ( 'NONE',  ( 21.36750515004459317, -279.2922091855626832, -221.7846871383528651 ) ) ;
#48410=CARTESIAN_POINT ( 'NONE',  ( 28.29141934333785002, -281.1877589585512851, -302.8008974023246651 ) ) ;
#48411=CARTESIAN_POINT ( 'NONE',  ( 34.84633991521791074, -279.2823340536546084, -249.3646139553059413 ) ) ;
#48412=CARTESIAN_POINT ( 'NONE',  ( -24.47571664943014014, -272.7941649313326025, -197.8533217057401714 ) ) ;
#48413=CARTESIAN_POINT ( 'NONE',  ( -111.5200163286703372, -280.6955736523474911, -259.2036772537322236 ) ) ;
#48416=CARTESIAN_POINT ( 'NONE',  ( -82.35206105707813151, -295.6874400992537062, -209.0745063143155846 ) ) ;
#48417=CARTESIAN_POINT ( 'NONE',  ( -111.6327960696554129, -290.8062707679650885, -250.0667521518485330 ) ) ;
#48418=CARTESIAN_POINT ( 'NONE',  ( 37.79750349199251502, -277.5262850201946208, -268.3292462118521939 ) ) ;
#48420=CARTESIAN_POINT ( 'NONE',  ( -108.6269844898742463, -286.7943788840112802, -245.3067285406265512 ) ) ;
#48423=CARTESIAN_POINT ( 'NONE',  ( 35.14691788232295266, -285.3023664409815865, -250.9209653761595575 ) ) ;
#48425=CARTESIAN_POINT ( 'NONE',  ( -2.971326231395900574, -293.3821643461020017, -335.2133184378173496 ) ) ;
#48426=CARTESIAN_POINT ( 'NONE',  ( 36.68162543543989784, -285.7727716755440497, -276.6084761632639015 ) ) ;
#48427=CARTESIAN_POINT ( 'NONE',  ( 202.9737475146022803, 296.4636489462809550, -68.70538243550777224 ) ) ;
#48428=CARTESIAN_POINT ( 'NONE',  ( 26.10596288904169526, -292.0908665098451706, -310.4510551253961808 ) ) ;
#48429=CARTESIAN_POINT ( 'NONE',  ( -89.39897259387291228, -283.8151017518756589, -214.4972623201564943 ) ) ;
#48430=CARTESIAN_POINT ( 'NONE',  ( -110.7641900578178706, -280.2559743114786102, -262.4149096979377305 ) ) ;
#48431=CARTESIAN_POINT ( 'NONE',  ( 0.07636131580060794011, -287.7438180743660041, -203.5038169974123718 ) ) ;
#48432=CARTESIAN_POINT ( 'NONE',  ( 12.34669393533375370, -278.9729366182945682, -212.8716623681657154 ) ) ;
#48433=CARTESIAN_POINT ( 'NONE',  ( -10.72409956425161859, -288.6952319305488572, -338.3896182484019164 ) ) ;
#48434=CARTESIAN_POINT ( 'NONE',  ( -81.65706671060000588, -280.8610423810284260, -211.5474554116948127 ) ) ;
#48435=CARTESIAN_POINT ( 'NONE',  ( -9.194650087268422922, -281.2326790994700332, -202.8307892314358014 ) ) ;
#48437=CARTESIAN_POINT ( 'NONE',  ( -46.33475724499292170, -287.9184698278778001, -195.5444639200435972 ) ) ;
#48440=CARTESIAN_POINT ( 'NONE',  ( -92.16906346390284455, -273.2947722073475916, -216.2967098230155045 ) ) ;
#48441=CARTESIAN_POINT ( 'NONE',  ( -101.7098150102609253, -292.0232716020706789, -308.2595933551771736 ) ) ;
#48443=CARTESIAN_POINT ( 'NONE',  ( -99.90806341382572953, -293.6948066931273047, -220.5068182859052968 ) ) ;
#48445=CARTESIAN_POINT ( 'NONE',  ( -62.90898176987437296, -271.7198730224327505, -199.6763067759649743 ) ) ;
#48448=CARTESIAN_POINT ( 'NONE',  ( -53.14345620473566356, -293.6512212790958074, -344.9586749577342744 ) ) ;
#48449=CARTESIAN_POINT ( 'NONE',  ( -36.47620041754861120, -297.5709263286453279, -197.2996537443671343 ) ) ;
#48450=CARTESIAN_POINT ( 'NONE',  ( -45.41940187598815726, -290.6764806551607876, -343.6104079885153624 ) ) ;
#48451=CARTESIAN_POINT ( 'NONE',  ( 26.44355838259787461, -283.8220636521855909, -308.0046169842578934 ) ) ;
#48452=CARTESIAN_POINT ( 'NONE',  ( -38.88990001302435218, -290.4964849865502856, -346.7562053372633954 ) ) ;
#48453=CARTESIAN_POINT ( 'NONE',  ( -111.4401933423845179, -291.6268495340742106, -289.4584695119689854 ) ) ;
#48454=CARTESIAN_POINT ( 'NONE',  ( -87.07080284692968064, -287.3602571608963103, -214.1488561749995370 ) ) ;
#48455=CARTESIAN_POINT ( 'NONE',  ( 3.820177922163388029, -280.7562482401743296, -205.2235664643215785 ) ) ;
#48456=CARTESIAN_POINT ( 'NONE',  ( -97.14993227689251398, -294.0039261174249532, -316.5378390554113253 ) ) ;
#48457=CARTESIAN_POINT ( 'NONE',  ( -83.88489227565895590, -283.5045877140880748, -331.7692036055802873 ) ) ;
#48458=CARTESIAN_POINT ( 'NONE',  ( 36.58621853088934017, -277.5001032749867704, -277.1085857651668789 ) ) ;
#48459=EDGE_CURVE ( 'NONE', #85436, #51665, #13474, .T. ) ;
#48460=CARTESIAN_POINT ( 'NONE',  ( 17.36665895637874613, -277.4090924074130839, -226.6919474004047572 ) ) ;
#48461=CARTESIAN_POINT ( 'NONE',  ( 34.23874395593382047, -274.1199092519049714, -296.0153740787582706 ) ) ;
#48463=CARTESIAN_POINT ( 'NONE',  ( 21.05531482523297981, -281.6760586903100716, -314.2882480912825827 ) ) ;
#48464=CARTESIAN_POINT ( 'NONE',  ( -64.93762771809339540, -278.6096719128904056, -341.8767019737751411 ) ) ;
#48465=CARTESIAN_POINT ( 'NONE',  ( -32.30983546127264816, -285.1728684155979749, -193.7483800310014317 ) ) ;
#48466=CARTESIAN_POINT ( 'NONE',  ( 29.64626065593770932, -294.8915279826618985, -238.7666438857950766 ) ) ;
#48467=CARTESIAN_POINT ( 'NONE',  ( -27.12417642901079873, -275.7799538497902745, -194.7963733936756512 ) ) ;
#48468=CARTESIAN_POINT ( 'NONE',  ( -93.79278064000719439, -274.5743418909764841, -218.7028914374340616 ) ) ;
#48470=CARTESIAN_POINT ( 'NONE',  ( -7.509593793271800877, -276.4830933680128169, -336.9872797822364987 ) ) ;
#48471=CARTESIAN_POINT ( 'NONE',  ( -110.3756934308333655, -298.3424059734609273, -286.6725941078428832 ) ) ;
#48472=CARTESIAN_POINT ( 'NONE',  ( -78.02491738921889919, -283.5042462350346568, -207.4911749699294887 ) ) ;
#48473=CARTESIAN_POINT ( 'NONE',  ( -5.891690441461046923, -292.1211023267514406, -200.0855977994165471 ) ) ;
#48474=CARTESIAN_POINT ( 'NONE',  ( 20.43913502912967317, -274.2268835606034258, -317.6382277688815634 ) ) ;
#48475=CARTESIAN_POINT ( 'NONE',  ( -2.151864020904867836, -290.1942795054138742, -337.9489560309091871 ) ) ;
#48477=CARTESIAN_POINT ( 'NONE',  ( -107.6880524943663460, -289.7448004320496580, -249.6860919924308178 ) ) ;
#48479=CARTESIAN_POINT ( 'NONE',  ( -66.77160279676913035, -290.2487522309768337, -199.8452536505324133 ) ) ;
#48480=CARTESIAN_POINT ( 'NONE',  ( -106.5899974854495724, -290.5264821146903387, -247.1930192287348120 ) ) ;
#48482=CARTESIAN_POINT ( 'NONE',  ( 38.47788378599893377, -288.4859750989545546, -258.7462869889035346 ) ) ;
#48483=CARTESIAN_POINT ( 'NONE',  ( -97.66390361071735526, -278.3130895153622646, -311.5110785389270518 ) ) ;
#48484=CARTESIAN_POINT ( 'NONE',  ( 19.29208684184133205, -293.1790951085636152, -322.1502179590457899 ) ) ;
#48485=CARTESIAN_POINT ( 'NONE',  ( -112.8996694329544539, -285.3859865675398169, -255.7903329040109952 ) ) ;
#48486=CARTESIAN_POINT ( 'NONE',  ( -37.98652757589916718, -286.3775594891009746, -193.3849626536423330 ) ) ;
#48487=CARTESIAN_POINT ( 'NONE',  ( -53.69027532592874508, -283.6009191893111847, -341.5807062375296823 ) ) ;
#48488=CARTESIAN_POINT ( 'NONE',  ( 174.1719164811267717, 243.3713473155254974, -179.7619469166268971 ) ) ;
#48489=CARTESIAN_POINT ( 'NONE',  ( 178.5843439615907187, 254.0915921303116818, -166.0334337346760663 ) ) ;
#48490=CARTESIAN_POINT ( 'NONE',  ( -98.92547009169517480, -245.9928705138712814, -331.3919335924819620 ) ) ;
#48491=CARTESIAN_POINT ( 'NONE',  ( 35.00286357884867527, -274.6047000715706190, -259.3741877010614303 ) ) ;
#48492=CARTESIAN_POINT ( 'NONE',  ( 34.19187683319228910, -274.6838856643095710, -286.4547810613709089 ) ) ;
#48493=CARTESIAN_POINT ( 'NONE',  ( -112.5463371017922753, -295.8565216530885209, -286.6027152311422697 ) ) ;
#48495=CARTESIAN_POINT ( 'NONE',  ( 139.7900897011093946, 178.0076021264288784, -238.7226697176948278 ) ) ;
#48496=CARTESIAN_POINT ( 'NONE',  ( 38.24585406340965221, -274.3899969387756528, -282.5177053876520290 ) ) ;
#48497=CARTESIAN_POINT ( 'NONE',  ( -21.74200613358737399, -276.0149943206727130, -198.0104195880617510 ) ) ;
#48499=CARTESIAN_POINT ( 'NONE',  ( -108.6744119391808567, -297.8558996268588430, -241.8551319269994906 ) ) ;
#48500=CARTESIAN_POINT ( 'NONE',  ( -23.76759780397865285, -289.3664951167810955, -342.2023603892083088 ) ) ;
#48501=CARTESIAN_POINT ( 'NONE',  ( -112.7322456164178845, -297.5418981753459207, -255.4467094823427828 ) ) ;
#48502=CARTESIAN_POINT ( 'NONE',  ( -95.52867704675838922, -297.7256810389183670, -219.9447052457241512 ) ) ;
#48503=CARTESIAN_POINT ( 'NONE',  ( 35.20717371541275753, -293.8315864005167555, -278.9084309542953974 ) ) ;
#48505=CARTESIAN_POINT ( 'NONE',  ( 37.71030135641018433, -277.5893913046390935, -279.5480825915715855 ) ) ;
#48506=CARTESIAN_POINT ( 'NONE',  ( 15.12395755914652717, -280.2763467993574409, -214.0132291253211179 ) ) ;
#48507=CARTESIAN_POINT ( 'NONE',  ( -80.94991160790036133, -278.6022145625182134, -329.1976061421860891 ) ) ;
#48508=CARTESIAN_POINT ( 'NONE',  ( 37.22003691802383685, -277.1266701044235106, -255.7145694236638747 ) ) ;
#48509=CARTESIAN_POINT ( 'NONE',  ( -69.61985833287917558, -275.4949673230672715, -338.4672990523591238 ) ) ;
#48510=CARTESIAN_POINT ( 'NONE',  ( -107.5595865702545950, -297.4720976119592137, -250.0303262631050529 ) ) ;
#48511=CARTESIAN_POINT ( 'NONE',  ( -92.64539109941854633, -294.4394483787563672, -318.9087923146258845 ) ) ;
#48513=CARTESIAN_POINT ( 'NONE',  ( 24.53851280884602915, -281.4363912407335420, -224.6405957821803554 ) ) ;
#48514=CARTESIAN_POINT ( 'NONE',  ( -3.865575368489865049, -276.7642761889835583, -335.2329075031861407 ) ) ;
#48516=CARTESIAN_POINT ( 'NONE',  ( 37.24265694736835997, -286.0218015860756964, -253.2596803548573519 ) ) ;
#48517=CARTESIAN_POINT ( 'NONE',  ( -26.56445917831958070, -300.1869189658202686, -195.1907785223500582 ) ) ;
#48518=CARTESIAN_POINT ( 'NONE',  ( 82.67621202554614968, -297.4092476797243307, -196.6572098816457128 ) ) ;
#48519=CARTESIAN_POINT ( 'NONE',  ( 8.072200834668189273, -287.6098455814253043, -327.7212027607546929 ) ) ;
#48520=CARTESIAN_POINT ( 'NONE',  ( -5.097046267291682753, -278.7224341710114004, -203.7408784592001609 ) ) ;
#48521=CARTESIAN_POINT ( 'NONE',  ( -51.92652732298921592, -278.4367009428111714, -198.1795208908974644 ) ) ;
#48522=CARTESIAN_POINT ( 'NONE',  ( -76.91292002685007390, -281.6660331980692149, -333.4731236785188457 ) ) ;
#48523=CARTESIAN_POINT ( 'NONE',  ( 37.67126975303213499, -289.5831405755807282, -272.7617249258289007 ) ) ;
#48524=CARTESIAN_POINT ( 'NONE',  ( -96.40344299156578245, -279.1495234529978688, -313.9578722329522975 ) ) ;
#48526=CARTESIAN_POINT ( 'NONE',  ( 23.18494719328650788, -294.9485837885573574, -226.0720040256993855 ) ) ;
#48527=CARTESIAN_POINT ( 'NONE',  ( -56.68796319367613989, -275.5379502510399448, -343.8980754507609277 ) ) ;
#48528=CARTESIAN_POINT ( 'NONE',  ( -24.30328498879935140, -277.5328323974271143, -342.3424154904254806 ) ) ;
#48529=CARTESIAN_POINT ( 'NONE',  ( 14.50778077475415984, -284.3248188407257544, -324.7822513295351996 ) ) ;
#48531=CARTESIAN_POINT ( 'NONE',  ( -109.4010151578765999, -292.1792126301169219, -293.2644311013637548 ) ) ;
#48532=CARTESIAN_POINT ( 'NONE',  ( -110.6491284464200504, -294.3477994234162338, -286.2643238697359038 ) ) ;
#48533=CARTESIAN_POINT ( 'NONE',  ( -97.44768269725072685, -284.3915695113563515, -222.4922378949848678 ) ) ;
#48535=CARTESIAN_POINT ( 'NONE',  ( -8.763707148622318144, -273.1187530463055282, -202.5975911649564694 ) ) ;
#48536=CARTESIAN_POINT ( 'NONE',  ( -37.52968995737902702, -290.1893948565007122, -196.1134975340727067 ) ) ;
#48539=CARTESIAN_POINT ( 'NONE',  ( -76.79406813884942551, -290.0143276955342344, -204.9838922623639235 ) ) ;
#48540=CARTESIAN_POINT ( 'NONE',  ( -108.5274800976382039, -285.8972967721289820, -289.8773481186418053 ) ) ;
#48541=CARTESIAN_POINT ( 'NONE',  ( 31.79942591476769920, -285.3822833631823528, -238.7148740462976093 ) ) ;
#48542=CARTESIAN_POINT ( 'NONE',  ( -108.3247488557336311, -285.7224689388157230, -289.8195149053919977 ) ) ;
#48543=CARTESIAN_POINT ( 'NONE',  ( -41.34195792098572042, -286.8033705861726617, -197.2965581104351998 ) ) ;
#48545=CARTESIAN_POINT ( 'NONE',  ( 35.86818148910214177, -295.7608560810044196, -288.2679181945184155 ) ) ;
#48546=CARTESIAN_POINT ( 'NONE',  ( 19.71648825643512737, -274.3143712625620196, -319.9153000638197000 ) ) ;
#48547=CARTESIAN_POINT ( 'NONE',  ( 35.70854587149006676, -275.5778372274126014, -245.9154365035611818 ) ) ;
#48548=CARTESIAN_POINT ( 'NONE',  ( 33.12884984009559020, -291.2784084006629541, -242.9544201776374734 ) ) ;
#48549=CARTESIAN_POINT ( 'NONE',  ( -111.8274409895666821, -278.3072764748673649, -289.9289303317952999 ) ) ;
#48550=CARTESIAN_POINT ( 'NONE',  ( -100.1028850609206557, -297.9839955258374289, -310.8646754240701284 ) ) ;
#48553=CARTESIAN_POINT ( 'NONE',  ( -109.4092864213582033, -283.4257270079277191, -255.9560325915904571 ) ) ;
#48554=CARTESIAN_POINT ( 'NONE',  ( -103.0293296677127870, -277.0333375170012573, -234.1653175139212237 ) ) ;
#48556=CARTESIAN_POINT ( 'NONE',  ( 37.22398974777998149, -274.2373383866365089, -286.6290596188400173 ) ) ;
#48557=CARTESIAN_POINT ( 'NONE',  ( -69.30346389650966898, -276.8326780654829236, -336.1194676859682318 ) ) ;
#48558=CARTESIAN_POINT ( 'NONE',  ( 21.89522449714161922, -295.6811020158600058, -314.1982542349576875 ) ) ;
#48559=CARTESIAN_POINT ( 'NONE',  ( -31.08520886551058737, -279.0496433150603366, -193.8733797925853253 ) ) ;
#48560=CARTESIAN_POINT ( 'NONE',  ( -80.28308419656772799, -296.5913547891394728, -329.6860367077647993 ) ) ;
#48561=CARTESIAN_POINT ( 'NONE',  ( -83.87191789193516911, -296.9909501468564486, -331.1587595875762418 ) ) ;
#48562=CARTESIAN_POINT ( 'NONE',  ( -84.07320627970419480, -297.2224491615630768, -214.2133381966015691 ) ) ;
#48563=CARTESIAN_POINT ( 'NONE',  ( -102.8835268438573394, -293.0387598443886645, -233.7952358678388691 ) ) ;
#48564=CARTESIAN_POINT ( 'NONE',  ( -40.81859718022990791, -286.1763649603586259, -193.3874638339882210 ) ) ;
#48565=CARTESIAN_POINT ( 'NONE',  ( 37.51159335903436443, -273.8448430344791404, -282.4068221268042862 ) ) ;
#48566=CARTESIAN_POINT ( 'NONE',  ( -5.628433901237086090, -288.4797803625827441, -340.5271264891952683 ) ) ;
#48567=CARTESIAN_POINT ( 'NONE',  ( -70.49298316036426115, -281.5928280043658560, -203.4676691104416477 ) ) ;
#48569=CARTESIAN_POINT ( 'NONE',  ( -68.86539035052989277, -284.6859499126771311, -204.2438406562552586 ) ) ;
#48571=CARTESIAN_POINT ( 'NONE',  ( -89.37944076373352686, -289.3196994197348886, -216.2791188411365795 ) ) ;
#48572=CARTESIAN_POINT ( 'NONE',  ( 193.8665746513534316, 275.1768195097669150, -123.9090917457166938 ) ) ;
#48573=CARTESIAN_POINT ( 'NONE',  ( -30.51929870519063570, -285.6482580331405643, -197.5679691028414595 ) ) ;
#48575=CARTESIAN_POINT ( 'NONE',  ( 37.91724765769303929, -282.6831987777285349, -285.4909227368766551 ) ) ;
#48577=CARTESIAN_POINT ( 'NONE',  ( -112.9038302107002778, -289.4401844526968830, -283.9700036400129193 ) ) ;
#48578=CARTESIAN_POINT ( 'NONE',  ( 36.89345403409696900, -282.9343461429411377, -253.1113499512093199 ) ) ;
#48579=CARTESIAN_POINT ( 'NONE',  ( -104.5344324371445595, -279.3908246714688062, -306.9457458526396181 ) ) ;
#48580=CARTESIAN_POINT ( 'NONE',  ( 35.70279637953220941, -281.3980658527124774, -271.3158764120159958 ) ) ;
#48581=CARTESIAN_POINT ( 'NONE',  ( -18.80118689711731506, -276.2909034945998314, -197.6350496608846186 ) ) ;
#48582=CARTESIAN_POINT ( 'NONE',  ( -79.47696455969719409, -295.6044586643631646, -334.8096981940573755 ) ) ;
#48583=CARTESIAN_POINT ( 'NONE',  ( -107.2422238976989064, -288.9156423444279653, -244.0274977234545304 ) ) ;
#48584=CARTESIAN_POINT ( 'NONE',  ( -35.79364542511192582, -296.9923055376416983, -197.0522957913235871 ) ) ;
#48587=CARTESIAN_POINT ( 'NONE',  ( 12.90637352302024787, -284.2642277782934457, -325.2832928299513924 ) ) ;
#48588=CARTESIAN_POINT ( 'NONE',  ( -101.4879127869722026, -295.7427776016064627, -305.2516738424444611 ) ) ;
#48589=CARTESIAN_POINT ( 'NONE',  ( -40.63297081429274016, -293.0913668607279305, -193.7277561580065992 ) ) ;
#48590=CARTESIAN_POINT ( 'NONE',  ( -86.99199381964908184, -284.4165389495634031, -324.0842638890283069 ) ) ;
#48591=CARTESIAN_POINT ( 'NONE',  ( 38.26246997598464361, -274.4431446383857178, -256.9882097258093268 ) ) ;
#48592=CARTESIAN_POINT ( 'NONE',  ( -113.0314947971882731, -291.0325923373216597, -284.0136592794058288 ) ) ;
#48593=CARTESIAN_POINT ( 'NONE',  ( -111.3241663741660545, -282.4840936314431019, -286.6981976738247226 ) ) ;
#48594=CARTESIAN_POINT ( 'NONE',  ( -96.37210939784807806, -290.2201101636690055, -319.7896087343793283 ) ) ;
#48595=CARTESIAN_POINT ( 'NONE',  ( 35.47333885171664036, -287.9661155069417191, -276.4788832650269796 ) ) ;
#48598=CARTESIAN_POINT ( 'NONE',  ( 153.5077555025204674, 204.5572234277026951, -214.3296801316302833 ) ) ;
#48599=CARTESIAN_POINT ( 'NONE',  ( -63.65460609925754909, -284.9091580461238777, -341.9875009121750509 ) ) ;
#48600=CARTESIAN_POINT ( 'NONE',  ( -106.6662871844225293, -287.6237833571633473, -303.7098442033569086 ) ) ;
#48602=CARTESIAN_POINT ( 'NONE',  ( 28.42231367664016517, -280.9109646802627935, -302.8694950075523025 ) ) ;
#48603=CARTESIAN_POINT ( 'NONE',  ( 3.486687757114208086, -276.1861857862203919, -335.6832454544615416 ) ) ;
#48604=CARTESIAN_POINT ( 'NONE',  ( -69.32950092992300029, -281.6304327545341266, -202.7090002712346575 ) ) ;
#48605=CARTESIAN_POINT ( 'NONE',  ( -110.6141395889435444, -273.5598078522675110, -270.3739478531805389 ) ) ;
#48606=CARTESIAN_POINT ( 'NONE',  ( 30.54527415402887414, -280.5824565906594330, -305.4319750315027022 ) ) ;
#48607=CARTESIAN_POINT ( 'NONE',  ( -108.0831924592627757, -282.8836220214131458, -246.3774263537814022 ) ) ;
#48608=CARTESIAN_POINT ( 'NONE',  ( -109.8263395877805806, -298.0214310851353616, -293.2070633060387763 ) ) ;
#48609=CARTESIAN_POINT ( 'NONE',  ( 18.51959070595551893, -293.3760210719144084, -223.2707301291225974 ) ) ;
#48611=CARTESIAN_POINT ( 'NONE',  ( -110.1136098019441221, -289.1012062508485769, -280.7225087094647620 ) ) ;
#48612=CARTESIAN_POINT ( 'NONE',  ( -11.89208267636104566, -277.3809297720416680, -342.9816323633611432 ) ) ;
#48613=CARTESIAN_POINT ( 'NONE',  ( -40.52009549172851166, -298.1777894119178995, -197.4177951610524815 ) ) ;
#48615=CARTESIAN_POINT ( 'NONE',  ( -69.98764049375895979, -272.5525468762258470, -200.9512658247716388 ) ) ;
#48619=CARTESIAN_POINT ( 'NONE',  ( 30.62624173263163385, -282.9981252987232665, -297.8308277024957533 ) ) ;
#48620=CARTESIAN_POINT ( 'NONE',  ( 36.00097875808192072, -283.0595617717870027, -250.4416142702418142 ) ) ;
#48621=CARTESIAN_POINT ( 'NONE',  ( -99.23629206093487198, -283.0705484777093375, -309.6028282686647231 ) ) ;
#48622=CARTESIAN_POINT ( 'NONE',  ( 21.48038547099317341, -282.7855586275067594, -225.0544016685380200 ) ) ;
#48623=CARTESIAN_POINT ( 'NONE',  ( 28.64276842741217166, -274.4741628800491071, -303.2900804249841826 ) ) ;
#48625=CARTESIAN_POINT ( 'NONE',  ( 32.81619808134219340, -276.9126943323491901, -291.6671964193691338 ) ) ;
#48628=CARTESIAN_POINT ( 'NONE',  ( -68.93960902322382367, -278.2599749774199154, -340.4164149230530825 ) ) ;
#48632=CARTESIAN_POINT ( 'NONE',  ( -109.7526578126973362, -286.6991158459916846, -247.8917827598084216 ) ) ;
#48634=CARTESIAN_POINT ( 'NONE',  ( 16.27052435803078723, -293.4632947254200985, -320.1439575232039942 ) ) ;
#48635=CARTESIAN_POINT ( 'NONE',  ( 7.867873377023919979, -287.8014451439553341, -332.6313369672537874 ) ) ;
#48636=CARTESIAN_POINT ( 'NONE',  ( -94.01680278720040462, -283.4587832512517025, -222.7595764697107938 ) ) ;
#48637=CARTESIAN_POINT ( 'NONE',  ( -105.7684773673082788, -282.7659416136862092, -297.5766785372172194 ) ) ;
#48638=CARTESIAN_POINT ( 'NONE',  ( -34.56209227983678289, -287.2567436409054267, -344.3725126396180940 ) ) ;
#48639=CARTESIAN_POINT ( 'NONE',  ( -102.1144633797219541, -285.2880576461042779, -304.9890918100404633 ) ) ;
#48640=CARTESIAN_POINT ( 'NONE',  ( -35.77939073807909409, -275.0324271141458894, -345.3576315030629758 ) ) ;
#48642=CARTESIAN_POINT ( 'NONE',  ( 22.37775995481749547, -285.3118579654935729, -223.0113948479123565 ) ) ;
#48643=CARTESIAN_POINT ( 'NONE',  ( -34.86830155287925948, -300.0832707502397056, -195.3602660063473877 ) ) ;
#48644=CARTESIAN_POINT ( 'NONE',  ( -32.40086865808414274, -284.1141308801414311, -195.3441546556174728 ) ) ;
#48645=CIRCLE ( 'NONE', #38090, 0.5000000000000004441 ) ;
#48646=CARTESIAN_POINT ( 'NONE',  ( 2.823044080410989309, -281.5466186746336348, -209.0613828178042581 ) ) ;
#48647=CARTESIAN_POINT ( 'NONE',  ( 34.63735439783157233, -289.8312778957915725, -292.0633002730257317 ) ) ;
#48648=CARTESIAN_POINT ( 'NONE',  ( 129.8975571001389540, -299.5541904835127980, -189.5200328990441676 ) ) ;
#48649=CARTESIAN_POINT ( 'NONE',  ( 115.2448031289451222, -299.5541904835127980, -195.3611179825600175 ) ) ;
#48650=CARTESIAN_POINT ( 'NONE',  ( -5.094472566048152018, -296.5511684722085306, -338.7085512838760337 ) ) ;
#48652=CARTESIAN_POINT ( 'NONE',  ( -98.00890200388300855, -277.1527077877407237, -226.2647318786002018 ) ) ;
#48653=CARTESIAN_POINT ( 'NONE',  ( -92.68866013613964583, -290.4812271823700485, -216.9855939435808523 ) ) ;
#48654=CARTESIAN_POINT ( 'NONE',  ( -87.04362444260598863, -294.1580886682608593, -324.9153032753341108 ) ) ;
#48655=CARTESIAN_POINT ( 'NONE',  ( -94.31226766204004264, -277.8897917451836292, -223.9327008822564835 ) ) ;
#48656=CARTESIAN_POINT ( 'NONE',  ( -72.56799164928743551, -271.6622520192747174, -204.7260835902301892 ) ) ;
#48657=CARTESIAN_POINT ( 'NONE',  ( 31.05059737066502734, -295.2263190217694842, -297.4028006318079633 ) ) ;
#48658=CARTESIAN_POINT ( 'NONE',  ( -95.95921662488163406, -298.4090924074130271, -317.1477375740089997 ) ) ;
#48659=CARTESIAN_POINT ( 'NONE',  ( -75.41700247900409693, -296.0343040350450110, -204.1719798737433962 ) ) ;
#48660=CARTESIAN_POINT ( 'NONE',  ( -16.87768598829033451, -290.5527697436305630, -197.1818986863124792 ) ) ;
#48661=CARTESIAN_POINT ( 'NONE',  ( -106.2688782327282553, -292.3202583836008444, -244.4401000466931464 ) ) ;
#48663=CARTESIAN_POINT ( 'NONE',  ( -64.14025613729464226, -292.4962417075998928, -202.2708391292083263 ) ) ;
#48665=CARTESIAN_POINT ( 'NONE',  ( -97.16315361736587874, -292.4014366067572723, -222.5134176920644791 ) ) ;
#48666=CARTESIAN_POINT ( 'NONE',  ( 28.31612186058764991, -280.0637668547256567, -307.4465468986252858 ) ) ;
#48667=CARTESIAN_POINT ( 'NONE',  ( 14.87550773271745008, -292.8133860569886906, -219.2753541556567995 ) ) ;
#48668=CARTESIAN_POINT ( 'NONE',  ( 30.72181242903524279, -281.0859349570575318, -234.2424698133636412 ) ) ;
#48669=CARTESIAN_POINT ( 'NONE',  ( -47.25784273800507407, -282.8415961742917375, -346.6986212637596623 ) ) ;
#48670=CARTESIAN_POINT ( 'NONE',  ( -72.04502145922313616, -287.5119327611447488, -336.6757324763734687 ) ) ;
#48671=CARTESIAN_POINT ( 'NONE',  ( -18.44368065994072126, -280.9458212278611313, -342.2038899071018250 ) ) ;
#48672=CARTESIAN_POINT ( 'NONE',  ( -56.36492323362677581, -278.2913641307645207, -196.4092236741880129 ) ) ;
#48673=CARTESIAN_POINT ( 'NONE',  ( -21.03623025897670828, -285.1769925888909825, -195.4236496424816778 ) ) ;
#48675=CARTESIAN_POINT ( 'NONE',  ( -5.717094902473006002, -294.0752255445763126, -203.6664197533825700 ) ) ;
#48676=CARTESIAN_POINT ( 'NONE',  ( 27.98926628453845922, -276.4549636358787552, -230.6308349732857153 ) ) ;
#48677=CARTESIAN_POINT ( 'NONE',  ( -32.42337306950857823, -276.6552935947437959, -343.2664181305506759 ) ) ;
#48678=CARTESIAN_POINT ( 'NONE',  ( -96.58022936636687916, -291.3804808366754742, -221.1493126920573502 ) ) ;
#48679=CARTESIAN_POINT ( 'NONE',  ( -34.55699062133827937, -281.0972555984808992, -345.8697902880177253 ) ) ;
#48680=CARTESIAN_POINT ( 'NONE',  ( 30.07703001190188630, -292.2265660479265534, -241.6284717467557925 ) ) ;
#48681=CARTESIAN_POINT ( 'NONE',  ( -111.1658611851397040, -294.7218451615552794, -257.1325921787241668 ) ) ;
#48683=CARTESIAN_POINT ( 'NONE',  ( 21.04675612459715950, -292.4436093660203255, -226.4432785746563468 ) ) ;
#48684=FACE_OUTER_BOUND ( 'NONE', #18906, .T. ) ;
#48685=CARTESIAN_POINT ( 'NONE',  ( -21.33282851196157992, -289.7666405000204009, -200.3683826091710216 ) ) ;
#48686=CARTESIAN_POINT ( 'NONE',  ( -112.0794853578401273, -295.3903608627329618, -287.9418139558929397 ) ) ;
#48687=CARTESIAN_POINT ( 'NONE',  ( 32.05127500298549847, -279.2975804070017602, -239.9486126536436643 ) ) ;
#48688=CARTESIAN_POINT ( 'NONE',  ( -2.462770587989639104, -287.8189127430741223, -202.2527129722085419 ) ) ;
#48689=CARTESIAN_POINT ( 'NONE',  ( 2.448791765869307024, -286.4353333299612814, -209.1588569186809536 ) ) ;
#48690=CARTESIAN_POINT ( 'NONE',  ( -32.35448218255530151, -278.5083975788343196, -343.9359449434364251 ) ) ;
#48691=CARTESIAN_POINT ( 'NONE',  ( -106.2716475864877879, -294.9479352107847490, -241.7165872052857196 ) ) ;
#48692=CARTESIAN_POINT ( 'NONE',  ( -110.1347373103682656, -298.1372364562573694, -283.8158207499173500 ) ) ;
#48694=CARTESIAN_POINT ( 'NONE',  ( -108.2076255699320200, -277.0960325370430155, -289.4700456591623947 ) ) ;
#48697=CARTESIAN_POINT ( 'NONE',  ( -107.1489830521686315, -295.8035128274034946, -302.8062646487720713 ) ) ;
#48698=CARTESIAN_POINT ( 'NONE',  ( -108.3178125325267018, -292.1785513154541150, -292.9748155868963408 ) ) ;
#48701=CARTESIAN_POINT ( 'NONE',  ( -31.85543656554987280, -289.6326526977358071, -343.3075840503252607 ) ) ;
#48703=CARTESIAN_POINT ( 'NONE',  ( -19.79831161777381610, -279.3309790245659201, -195.5733223984542235 ) ) ;
#48704=CARTESIAN_POINT ( 'NONE',  ( -95.49896296905055237, -296.5230147947148680, -320.6706157507477428 ) ) ;
#48705=CARTESIAN_POINT ( 'NONE',  ( -72.83377190921757460, -289.7267650075502274, -203.4090383468069660 ) ) ;
#48706=CARTESIAN_POINT ( 'NONE',  ( -111.6028049752585787, -297.1416555585039987, -249.8901708905887062 ) ) ;
#48708=CARTESIAN_POINT ( 'NONE',  ( 21.34599126082868992, -294.4944530964592104, -313.8104259894918755 ) ) ;
#48712=CARTESIAN_POINT ( 'NONE',  ( 23.60026902073524724, -289.6892833505908698, -316.2826178583721344 ) ) ;
#48713=CARTESIAN_POINT ( 'NONE',  ( 40.65961533371913106, -284.2662352645559167, -288.1317622949166548 ) ) ;
#48714=ORIENTED_EDGE ( 'NONE', *, *, #37168, .T. ) ;
#48716=CARTESIAN_POINT ( 'NONE',  ( 17.15673458860114309, -280.1530075973298040, -216.0348683170665254 ) ) ;
#48717=CARTESIAN_POINT ( 'NONE',  ( -112.0604175095280368, -286.6165758692659438, -265.3676268376449343 ) ) ;
#48718=CARTESIAN_POINT ( 'NONE',  ( 39.11262168029700348, -286.1419939503098817, -271.5602958330769070 ) ) ;
#48719=CARTESIAN_POINT ( 'NONE',  ( -84.32226885479330747, -271.4038055219076000, -212.1129026839008702 ) ) ;
#48720=CARTESIAN_POINT ( 'NONE',  ( -84.11398248106308984, -275.3234891689962183, -212.4502571845264640 ) ) ;
#48722=CARTESIAN_POINT ( 'NONE',  ( -91.79622353690605507, -289.3479024907310304, -219.5877803274311191 ) ) ;
#48723=CARTESIAN_POINT ( 'NONE',  ( -51.06525538948874754, -279.0861702300503566, -344.8726574175473729 ) ) ;
#48724=CARTESIAN_POINT ( 'NONE',  ( -93.09020038426017152, -279.2221087320643278, -223.2132920592192136 ) ) ;
#48725=CARTESIAN_POINT ( 'NONE',  ( -7.950860760758045487, -279.7962448637267698, -203.4140914288397823 ) ) ;
#48726=CARTESIAN_POINT ( 'NONE',  ( -2.851758475184907216, -277.6867484368544297, -338.8734492916458407 ) ) ;
#48727=CARTESIAN_POINT ( 'NONE',  ( -94.65446285177091568, -278.0392945534433125, -219.5353769835632818 ) ) ;
#48728=CARTESIAN_POINT ( 'NONE',  ( -32.42903041750177806, -123.8281167454940999, -361.7435837593322390 ) ) ;
#48729=CARTESIAN_POINT ( 'NONE',  ( -41.19299589062352140, -274.9461739899020358, -193.6409824334107839 ) ) ;
#48730=CARTESIAN_POINT ( 'NONE',  ( -102.1405766910263964, -274.6042108955197705, -230.0645505358623097 ) ) ;
#48731=CARTESIAN_POINT ( 'NONE',  ( -110.4683760289727132, -293.2662352645559167, -253.7030783399848985 ) ) ;
#48733=CARTESIAN_POINT ( 'NONE',  ( 82.64126209800332390, -300.1542085700246503, -192.9280458966490528 ) ) ;
#48734=CARTESIAN_POINT ( 'NONE',  ( 25.20733400835214155, -288.1072502891944396, -232.1270441503878033 ) ) ;
#48735=CARTESIAN_POINT ( 'NONE',  ( 36.16985707124061378, -289.5562826470426216, -289.5971512037937714 ) ) ;
#48736=CARTESIAN_POINT ( 'NONE',  ( 34.85859135095023476, -287.0525672471521261, -281.8868190740270734 ) ) ;
#48737=CARTESIAN_POINT ( 'NONE',  ( -76.73178316510245622, -283.0718821535951406, -336.5133457140380528 ) ) ;
#48738=CARTESIAN_POINT ( 'NONE',  ( -59.95964621383821935, -278.1541272356391801, -200.0586118444897465 ) ) ;
#48739=CARTESIAN_POINT ( 'NONE',  ( -5.286379073223693048, -288.3388638479190149, -203.3894899003055343 ) ) ;
#48740=CARTESIAN_POINT ( 'NONE',  ( 34.61324238663527098, -280.2399601952778312, -286.2731889461723540 ) ) ;
#48741=CARTESIAN_POINT ( 'NONE',  ( -91.67260161652997397, -280.5722119163197590, -220.8697387136645318 ) ) ;
#48742=CARTESIAN_POINT ( 'NONE',  ( -16.35720136710627415, -277.2659766378330346, -340.3973085479157135 ) ) ;
#48743=CARTESIAN_POINT ( 'NONE',  ( -37.51616981767915604, -287.8491851459787654, -346.9768523904389781 ) ) ;
#48744=CARTESIAN_POINT ( 'NONE',  ( -66.50547387911690578, -284.2273124513799303, -341.4641831580120197 ) ) ;
#48745=CARTESIAN_POINT ( 'NONE',  ( -108.1680342657487301, -284.6601246523491113, -300.5499602784155968 ) ) ;
#48746=CARTESIAN_POINT ( 'NONE',  ( -1.250160080634530324, -282.7256401586120660, -333.8150441141625038 ) ) ;
#48750=CARTESIAN_POINT ( 'NONE',  ( -110.4473060167651681, -292.6663860667849235, -250.4152013358639124 ) ) ;
#48751=CARTESIAN_POINT ( 'NONE',  ( 22.73133772193494906, -291.5990471942290014, -222.9637230989866623 ) ) ;
#48752=CARTESIAN_POINT ( 'NONE',  ( -8.868317561797425697, -273.4926146706915802, -202.8335151676897681 ) ) ;
#48753=CARTESIAN_POINT ( 'NONE',  ( 8.838316208477916547, -293.7858326752867697, -331.8486685715480462 ) ) ;
#48754=CARTESIAN_POINT ( 'NONE',  ( -87.21269467351521598, -288.2417882476885893, -324.6852384590505380 ) ) ;
#48755=CARTESIAN_POINT ( 'NONE',  ( 35.31491773729234751, -291.9755473941751802, -284.4674958264220663 ) ) ;
#48756=CARTESIAN_POINT ( 'NONE',  ( -96.87172919699636964, -291.1600270849020262, -313.2948593123961700 ) ) ;
#48758=CARTESIAN_POINT ( 'NONE',  ( -81.65004257335596094, -291.6555331179454811, -330.8736905244816171 ) ) ;
#48759=CARTESIAN_POINT ( 'NONE',  ( 33.72776378554834764, -291.2341105423036538, -245.7256645272244384 ) ) ;
#48760=CARTESIAN_POINT ( 'NONE',  ( 6.717849444255739044, -294.6510772731249972, -209.6039066691162702 ) ) ;
#48761=CARTESIAN_POINT ( 'NONE',  ( 16.13812384942448475, -287.7757202324366403, -220.3094575983584207 ) ) ;
#48762=CARTESIAN_POINT ( 'NONE',  ( 34.62208415254949045, -295.8334690835096126, -292.2457552112653616 ) ) ;
#48763=CARTESIAN_POINT ( 'NONE',  ( 20.57027291757417231, -276.8693526485226357, -222.1469065468835709 ) ) ;
#48764=CARTESIAN_POINT ( 'NONE',  ( -33.33465842890517905, -297.2982953954544314, -193.5231230048669886 ) ) ;
#48765=CARTESIAN_POINT ( 'NONE',  ( -9.629465080767708685, -274.9249340678638873, -339.0043537721063558 ) ) ;
#48766=CARTESIAN_POINT ( 'NONE',  ( -4.909440609980757486, -278.5624472350443739, -203.3576647534698907 ) ) ;
#48767=CARTESIAN_POINT ( 'NONE',  ( -94.09514317038249942, -274.4131280210744421, -223.7992525931428531 ) ) ;
#48768=CARTESIAN_POINT ( 'NONE',  ( 22.30983858929492314, -273.4821179802898996, -222.5878733686120654 ) ) ;
#48769=CARTESIAN_POINT ( 'NONE',  ( -110.9641573957463692, -297.9986740797583025, -268.7378648852824767 ) ) ;
#48771=CARTESIAN_POINT ( 'NONE',  ( -106.8634283265061953, -297.6586798984685629, -247.4116025793694007 ) ) ;
#48774=CARTESIAN_POINT ( 'NONE',  ( 36.41883083574412439, -285.3744006158579509, -254.8780723520905838 ) ) ;
#48775=CARTESIAN_POINT ( 'NONE',  ( -47.27274760131920317, -297.9225879078319394, -197.9885806972592661 ) ) ;
#48777=CARTESIAN_POINT ( 'NONE',  ( -43.66626749914844652, -285.9744620146761918, -193.5680395735372201 ) ) ;
#48778=CARTESIAN_POINT ( 'NONE',  ( -93.58025189592885340, -289.5011897254220230, -323.0019022192084321 ) ) ;
#48779=CARTESIAN_POINT ( 'NONE',  ( -96.08044335633468336, -299.1784132186828629, -223.1576556985411344 ) ) ;
#48780=CARTESIAN_POINT ( 'NONE',  ( -20.45871956450569229, -292.8348034763471901, -343.3185278757484866 ) ) ;
#48781=CARTESIAN_POINT ( 'NONE',  ( 20.01497926838791130, -280.0544944302019985, -219.2104189070933273 ) ) ;
#48782=CARTESIAN_POINT ( 'NONE',  ( 35.78497577281001440, -284.8380690714490129, -253.7030783399848985 ) ) ;
#48783=AXIS2_PLACEMENT_3D ( 'NONE', #72458, #21, #22259 ) ;
#48784=CARTESIAN_POINT ( 'NONE',  ( -10.59362080976867482, -287.4903506443534411, -338.7652451165742491 ) ) ;
#48786=CARTESIAN_POINT ( 'NONE',  ( -64.57010964823807342, -287.4072960800537544, -340.2996576680407657 ) ) ;
#48787=CARTESIAN_POINT ( 'NONE',  ( -101.3293075261046710, -274.5696475339431686, -233.7031034039917472 ) ) ;
#48788=CARTESIAN_POINT ( 'NONE',  ( 22.40315372552599271, -282.3344857988484478, -222.7046354972477502 ) ) ;
#48789=CARTESIAN_POINT ( 'NONE',  ( -112.1155930067112649, -270.7750857621161913, -259.1340169022741975 ) ) ;
#48790=CARTESIAN_POINT ( 'NONE',  ( 33.32351073033067479, -281.7945278179896604, -288.7256019913251635 ) ) ;
#48791=CARTESIAN_POINT ( 'NONE',  ( -97.40610338847450578, -296.0730728061060972, -318.5615180661544628 ) ) ;
#48792=CARTESIAN_POINT ( 'NONE',  ( -35.14096886606251502, -299.6003140158371707, -196.6671976274662370 ) ) ;
#48793=CARTESIAN_POINT ( 'NONE',  ( 30.20875484378765208, -283.1217076874604572, -237.6543525513209829 ) ) ;
#48794=CARTESIAN_POINT ( 'NONE',  ( 52.04239232965979767, -298.2568191073556818, -197.1405908929531847 ) ) ;
#48796=CARTESIAN_POINT ( 'NONE',  ( -98.72252273868838301, -287.1110187090874319, -227.8621508393838440 ) ) ;
#48798=CARTESIAN_POINT ( 'NONE',  ( -115.3430155898818299, -275.8380690714489560, -288.1317622949166548 ) ) ;
#48799=CARTESIAN_POINT ( 'NONE',  ( 35.04539715609341499, -275.0770636427558316, -296.2912665264293537 ) ) ;
#48801=CARTESIAN_POINT ( 'NONE',  ( -94.81367959793740852, -285.4263216955772009, -316.5079593686362500 ) ) ;
#48803=CARTESIAN_POINT ( 'NONE',  ( 21.48683435282068643, -277.7716642127030582, -314.9216829241832443 ) ) ;
#48805=CARTESIAN_POINT ( 'NONE',  ( -78.82449837061346898, -285.0247907745338694, -334.5310777917760561 ) ) ;
#48806=CARTESIAN_POINT ( 'NONE',  ( -91.04238729555980569, -282.6314891182660745, -320.3947736833543445 ) ) ;
#48807=CARTESIAN_POINT ( 'NONE',  ( 8.340899652445068924, -282.6770541029541732, -210.8134886029699260 ) ) ;
#48808=CARTESIAN_POINT ( 'NONE',  ( -70.13369836670366908, -273.7986963956612385, -200.6783123985541408 ) ) ;
#48809=CARTESIAN_POINT ( 'NONE',  ( 31.85435142406308628, -275.8205306064180036, -304.2598640022296763 ) ) ;
#48811=CARTESIAN_POINT ( 'NONE',  ( -69.11009981657500134, -297.3933657055421236, -337.6958654890304956 ) ) ;
#48815=CARTESIAN_POINT ( 'NONE',  ( -101.2613947813466098, -295.2336151009571950, -229.6846122945249249 ) ) ;
#48816=CARTESIAN_POINT ( 'NONE',  ( 3.163017461392574337, -275.9992441355225878, -331.1670082773658805 ) ) ;
#48817=CARTESIAN_POINT ( 'NONE',  ( -71.66782037961642970, -287.3521951186393153, -204.7890851943573693 ) ) ;
#48818=CARTESIAN_POINT ( 'NONE',  ( 38.13364687008371590, -295.2140308440156673, -281.5940939132642598 ) ) ;
#48819=CARTESIAN_POINT ( 'NONE',  ( 30.53990758182080967, -294.2955605422340568, -234.7491367700766318 ) ) ;
#48820=CARTESIAN_POINT ( 'NONE',  ( -112.2024507298690139, -292.5770464885447950, -268.4394741229540955 ) ) ;
#48821=CARTESIAN_POINT ( 'NONE',  ( -111.9993164492161952, -276.4768869494644150, -276.1971161971118818 ) ) ;
#48822=CARTESIAN_POINT ( 'NONE',  ( -71.62622501710009715, -281.5157508758462654, -204.2719024443072726 ) ) ;
#48823=CARTESIAN_POINT ( 'NONE',  ( -45.26790214284979896, -293.2330298569958131, -344.4294100322289296 ) ) ;
#48824=CARTESIAN_POINT ( 'NONE',  ( -64.78237100356091105, -285.2671086301278365, -340.9960170492306020 ) ) ;
#48825=CARTESIAN_POINT ( 'NONE',  ( -110.6998422714887624, -283.4654230564982527, -270.8978990543860164 ) ) ;
#48826=CARTESIAN_POINT ( 'NONE',  ( 169.7661770085315140, 230.6591521943099110, -191.8278467606775450 ) ) ;
#48828=CARTESIAN_POINT ( 'NONE',  ( -81.48798803269406221, -285.0990964972142478, -212.1958985561396958 ) ) ;
#48830=CARTESIAN_POINT ( 'NONE',  ( 38.56727514591051431, -282.7689826971383127, -281.2844866282564453 ) ) ;
#48832=CARTESIAN_POINT ( 'NONE',  ( -97.26016824723730281, -283.9893914948825113, -222.6349626906605579 ) ) ;
#48833=CARTESIAN_POINT ( 'NONE',  ( -107.2099568342708267, -279.9025493815156551, -238.4329833986973881 ) ) ;
#48835=CARTESIAN_POINT ( 'NONE',  ( -23.04960382704055988, -278.3927875219746397, -345.3710959646958258 ) ) ;
#48836=CARTESIAN_POINT ( 'NONE',  ( -11.55136634270433227, -281.0306925004511527, -197.8609480248495913 ) ) ;
#48837=CARTESIAN_POINT ( 'NONE',  ( -37.37352853689063181, -300.5519495502701375, -200.3611179825600459 ) ) ;
#48838=CARTESIAN_POINT ( 'NONE',  ( 190.8961174813688615, 270.6925287644853029, -139.5879506144360676 ) ) ;
#48840=CARTESIAN_POINT ( 'NONE',  ( 3.920097784138138142, -276.6089133133280598, -207.8693004201030590 ) ) ;
#48841=CARTESIAN_POINT ( 'NONE',  ( -64.29435065518906356, -182.4202019385718643, -362.1134662045771506 ) ) ;
#48843=CARTESIAN_POINT ( 'NONE',  ( -109.5575993125019210, -276.8167122651744876, -251.4241912110171029 ) ) ;
#48844=CARTESIAN_POINT ( 'NONE',  ( 37.06501242101278848, -295.1161266534670062, -254.8826641732230769 ) ) ;
#48845=CARTESIAN_POINT ( 'NONE',  ( -7.954933637996020046, -294.0052857975274492, -337.3098359824493286 ) ) ;
#48846=CARTESIAN_POINT ( 'NONE',  ( -113.7532073829613211, -289.9417846639206005, -279.7905033142632192 ) ) ;
#48849=CARTESIAN_POINT ( 'NONE',  ( -64.07715268106635165, -293.9689222698381172, -341.9419944045560555 ) ) ;
#48850=CARTESIAN_POINT ( 'NONE',  ( -46.80750696547797673, -284.3299768624214607, -197.1193578559215496 ) ) ;
#48851=CARTESIAN_POINT ( 'NONE',  ( -63.25370804099521393, -293.5713874822761795, -200.7950822612816921 ) ) ;
#48852=CARTESIAN_POINT ( 'NONE',  ( -46.79480603712902820, -284.4099703930809824, -197.2253447062450675 ) ) ;
#48853=CARTESIAN_POINT ( 'NONE',  ( -108.2324381847122226, -285.6123884490899627, -289.7927781901291269 ) ) ;
#48855=CARTESIAN_POINT ( 'NONE',  ( -37.80567232658941634, -292.9877206998336874, -193.5978133120024154 ) ) ;
#48857=CARTESIAN_POINT ( 'NONE',  ( 3.429756406300124016, -282.9802314699958856, -331.0496782240537073 ) ) ;
#48858=CARTESIAN_POINT ( 'NONE',  ( -88.35251561539841703, -294.5428128083704564, -327.5803626996567459 ) ) ;
#48859=CARTESIAN_POINT ( 'NONE',  ( -109.7100097668032674, -291.0265331231349819, -296.3448835064751847 ) ) ;
#48860=CARTESIAN_POINT ( 'NONE',  ( -80.50090365319508123, -290.1121457277528179, -334.1185680935244591 ) ) ;
#48861=CARTESIAN_POINT ( 'NONE',  ( 35.55250553501682731, -287.6558229110160028, -265.5845879727958732 ) ) ;
#48864=CARTESIAN_POINT ( 'NONE',  ( -111.3927971968902142, -298.2089040087636249, -286.3842421237368967 ) ) ;
#48866=CARTESIAN_POINT ( 'NONE',  ( -9.318050067021886207, -297.0809218362947490, -193.8603748128029736 ) ) ;
#48867=CARTESIAN_POINT ( 'NONE',  ( -76.93903086589591567, -278.5665362596325281, -208.6933674503681289 ) ) ;
#48869=CARTESIAN_POINT ( 'NONE',  ( 36.82462404239806375, -275.3169603148791680, -290.8768648620383601 ) ) ;
#48870=CARTESIAN_POINT ( 'NONE',  ( -94.13562889880033424, -295.6916931295959898, -223.3823892766719723 ) ) ;
#48871=CARTESIAN_POINT ( 'NONE',  ( 26.25761974421145339, -277.8256077703858296, -308.2174321690018814 ) ) ;
#48872=CARTESIAN_POINT ( 'NONE',  ( -13.64916646131800526, -272.5025748830576617, -200.0082265890458473 ) ) ;
#48873=CARTESIAN_POINT ( 'NONE',  ( -38.33234156308011364, -296.2699215360458425, -343.7515065605587665 ) ) ;
#48874=CARTESIAN_POINT ( 'NONE',  ( -20.76496692736728633, -295.9141398178044255, -341.8237951098844860 ) ) ;
#48876=CARTESIAN_POINT ( 'NONE',  ( -58.60830574555028960, -296.9226618092444596, -343.5883154043546597 ) ) ;
#48878=CARTESIAN_POINT ( 'NONE',  ( -36.88444583258380760, -296.0577074479207909, -195.1945980807678325 ) ) ;
#48879=CARTESIAN_POINT ( 'NONE',  ( -52.39885591807911425, -292.5057482764098040, -198.7747129985252741 ) ) ;
#48880=CARTESIAN_POINT ( 'NONE',  ( -68.78735336093448893, -274.4520380518480920, -200.2373395437965939 ) ) ;
#48881=CARTESIAN_POINT ( 'NONE',  ( -105.6668342468205140, -288.7623754021108198, -297.8301995730903400 ) ) ;
#48883=CARTESIAN_POINT ( 'NONE',  ( -110.9800606624915815, -273.3265990528932434, -247.8872775669179589 ) ) ;
#48885=CARTESIAN_POINT ( 'NONE',  ( -107.9889556372695552, -296.6410895767857028, -288.8781580677458578 ) ) ;
#48887=CARTESIAN_POINT ( 'NONE',  ( -50.67392717452807460, -281.8625606862206610, -196.1946934897722770 ) ) ;
#48888=CARTESIAN_POINT ( 'NONE',  ( 38.92147502931899083, -280.1601826203132077, -264.2597749594601169 ) ) ;
#48889=CARTESIAN_POINT ( 'NONE',  ( -11.90773598810970846, -276.0783133199085455, -342.9871152434971009 ) ) ;
#48890=CARTESIAN_POINT ( 'NONE',  ( 38.84169934355085019, -279.9109634800678350, -267.1120261466754755 ) ) ;
#48891=CARTESIAN_POINT ( 'NONE',  ( 32.86582971841230716, -279.9002235044725353, -297.2112795726115451 ) ) ;
#48892=CARTESIAN_POINT ( 'NONE',  ( -74.55581212949162762, -272.1217423160327940, -206.8159976636424062 ) ) ;
#48893=CARTESIAN_POINT ( 'NONE',  ( -18.58858278732690295, -278.8109108328932848, -343.0316977440042479 ) ) ;
#48896=CARTESIAN_POINT ( 'NONE',  ( -31.97581412555593161, -296.3583192041082839, -194.3760267278788092 ) ) ;
#48897=CARTESIAN_POINT ( 'NONE',  ( -13.86645436775929596, -292.3484273333282886, -196.9708888462583900 ) ) ;
#48898=CARTESIAN_POINT ( 'NONE',  ( 35.46937008295187610, -277.7916533625960369, -289.0313211020973085 ) ) ;
#48899=CARTESIAN_POINT ( 'NONE',  ( -72.83225659644364214, -271.5822585212394529, -204.2319261592077737 ) ) ;
#48901=CARTESIAN_POINT ( 'NONE',  ( 27.09011957082900324, -283.9989411684799734, -309.9299922774285960 ) ) ;
#48903=CARTESIAN_POINT ( 'NONE',  ( -5.239512184654298466, -284.4743694816795596, -202.5648510644412568 ) ) ;
#48905=CARTESIAN_POINT ( 'NONE',  ( -5.382408334676391348, -293.4169320221702151, -336.4487045733047239 ) ) ;
#48906=CARTESIAN_POINT ( 'NONE',  ( 15.93214297801810098, -284.9567541479334523, -218.6623450708501082 ) ) ;
#48908=CARTESIAN_POINT ( 'NONE',  ( 20.35582022997981611, -292.2135310197681974, -318.2776787626873443 ) ) ;
#48909=CARTESIAN_POINT ( 'NONE',  ( -69.48300058784650446, -284.1167174138755627, -201.1396252506790745 ) ) ;
#48910=CARTESIAN_POINT ( 'NONE',  ( -38.38542137872376969, -281.6389881503830566, -196.5559589294611840 ) ) ;
#48911=CARTESIAN_POINT ( 'NONE',  ( -23.87089300761373423, -287.4255132498776106, -194.8979917461260811 ) ) ;
#48912=CARTESIAN_POINT ( 'NONE',  ( 20.31208404138603285, -279.1148563649746848, -220.8436973572415525 ) ) ;
#48913=CARTESIAN_POINT ( 'NONE',  ( 27.65814003892320017, -287.0993824648368218, -237.0228571196263658 ) ) ;
#48914=VECTOR ( 'NONE', #24422, 1000.000000000000000 ) ;
#48915=CARTESIAN_POINT ( 'NONE',  ( -66.31829895787133466, -281.0904749840060504, -202.7032126429618586 ) ) ;
#48916=CARTESIAN_POINT ( 'NONE',  ( 17.17633097946117715, -281.6584852969534154, -221.5719182415239459 ) ) ;
#48917=CARTESIAN_POINT ( 'NONE',  ( -67.85827863381908287, -287.6335187730401799, -201.4475162250844278 ) ) ;
#48921=CARTESIAN_POINT ( 'NONE',  ( -98.23266610948735433, -297.0149026693531482, -223.2092732495960945 ) ) ;
#48922=CARTESIAN_POINT ( 'NONE',  ( -92.91419131404576603, -293.2296722294915412, -220.5068134914450297 ) ) ;
#48924=CARTESIAN_POINT ( 'NONE',  ( -72.08107566293803359, -300.1233781216987495, -198.2974183793908196 ) ) ;
#48926=CARTESIAN_POINT ( 'NONE',  ( -80.18403987036899139, -271.4738533065243473, -208.5359152840082402 ) ) ;
#48928=CARTESIAN_POINT ( 'NONE',  ( -105.2540632708972765, -294.5010128878602700, -305.0368010975247444 ) ) ;
#48929=CARTESIAN_POINT ( 'NONE',  ( -60.52949302720537617, -297.2509154886362239, -201.0233020330287559 ) ) ;
#48931=CARTESIAN_POINT ( 'NONE',  ( 4.019609066241355499, -290.0042790554126668, -331.4140517803542139 ) ) ;
#48932=CARTESIAN_POINT ( 'NONE',  ( 22.92578535756121383, -282.7203185387714370, -227.3982944264695618 ) ) ;
#48933=CARTESIAN_POINT ( 'NONE',  ( -112.0799808880328925, -291.6614590135502567, -286.7161680874208400 ) ) ;
#48934=CARTESIAN_POINT ( 'NONE',  ( 10.28133781032519956, -288.7094029330172020, -212.4210894774008409 ) ) ;
#48935=CARTESIAN_POINT ( 'NONE',  ( -31.07587571008332716, -280.2957936943342929, -193.5637893441634958 ) ) ;
#48936=CARTESIAN_POINT ( 'NONE',  ( -37.70702677364511857, -293.1365090615122995, -345.9330722352666498 ) ) ;
#48937=CARTESIAN_POINT ( 'NONE',  ( 39.64073502675631744, -281.3441811152776495, -267.0594941863539020 ) ) ;
#48939=CARTESIAN_POINT ( 'NONE',  ( 20.80852366203457748, -276.7717962356991848, -224.1951808642405126 ) ) ;
#48940=CARTESIAN_POINT ( 'NONE',  ( -21.39648532958013050, -276.7662352645559167, -200.3538533559491555 ) ) ;
#48941=CARTESIAN_POINT ( 'NONE',  ( 36.25166463110930692, -274.0319597747138687, -289.2817596117944277 ) ) ;
#48943=CARTESIAN_POINT ( 'NONE',  ( 31.13017105736646783, -280.7184194820921448, -244.7288588045542781 ) ) ;
#48945=CARTESIAN_POINT ( 'NONE',  ( -59.53523291736747325, -278.5384208520371203, -343.6786180763897391 ) ) ;
#48946=CARTESIAN_POINT ( 'NONE',  ( -83.51331696775213231, -274.7186064872564089, -213.1822296148037879 ) ) ;
#48947=CARTESIAN_POINT ( 'NONE',  ( -110.6976144103448121, -283.8978999627197481, -247.5608459168789182 ) ) ;
#48948=CARTESIAN_POINT ( 'NONE',  ( -94.23293937510810281, -292.9749340288964277, -222.9983115447663522 ) ) ;
#48949=CARTESIAN_POINT ( 'NONE',  ( -94.50002868054474447, -274.8417268522022141, -219.9689966385420519 ) ) ;
#48950=CARTESIAN_POINT ( 'NONE',  ( -112.5863935297308700, -274.0450845658967296, -256.2383464419285701 ) ) ;
#48952=CARTESIAN_POINT ( 'NONE',  ( 19.18024537832320675, -276.0398022582805311, -316.5789716663322793 ) ) ;
#48953=CARTESIAN_POINT ( 'NONE',  ( -89.76852189558813677, -297.7936146566669890, -323.8329496689507323 ) ) ;
#48954=CARTESIAN_POINT ( 'NONE',  ( -86.92223003320941643, -283.3605800723489097, -214.2401237080880492 ) ) ;
#48955=CARTESIAN_POINT ( 'NONE',  ( -42.04842835355492525, -291.6610673955120205, -193.5262886344245601 ) ) ;
#48956=CARTESIAN_POINT ( 'NONE',  ( 25.35245526591383580, -274.1218991087860104, -310.9692089050035975 ) ) ;
#48957=CARTESIAN_POINT ( 'NONE',  ( 38.90232380747248442, -289.1669077958005687, -271.5185865521456776 ) ) ;
#48959=CARTESIAN_POINT ( 'NONE',  ( -49.72747728650247723, -290.8109238110834553, -198.0543438882310170 ) ) ;
#48960=ORIENTED_EDGE ( 'NONE', *, *, #78765, .F. ) ;
#48961=CARTESIAN_POINT ( 'NONE',  ( 21.76509671230398979, -291.4716276612833212, -221.9359916285157794 ) ) ;
#48963=CARTESIAN_POINT ( 'NONE',  ( -104.0687647103991225, -289.8182357120257961, -300.1438274952589040 ) ) ;
#48965=CARTESIAN_POINT ( 'NONE',  ( 14.02958246012962995, -287.8326412374968299, -213.3470710461920703 ) ) ;
#48966=CARTESIAN_POINT ( 'NONE',  ( -109.5123143934463741, -278.7388836678495068, -281.4737199890546435 ) ) ;
#48967=CARTESIAN_POINT ( 'NONE',  ( 10.99279277905546515, -293.3218042508020744, -329.9717075471970134 ) ) ;
#48968=CARTESIAN_POINT ( 'NONE',  ( -33.74041141479603567, -286.7477657199906389, -193.5474245002785381 ) ) ;
#48969=CARTESIAN_POINT ( 'NONE',  ( -110.9070844177439454, -285.1722274901824221, -247.5127842735608397 ) ) ;
#48970=CARTESIAN_POINT ( 'NONE',  ( 33.67170838645847653, -282.1104001074387497, -287.4197168481941844 ) ) ;
#48971=CARTESIAN_POINT ( 'NONE',  ( -71.22237285446017552, -196.1705862519446839, -360.4586094979653126 ) ) ;
#48972=CARTESIAN_POINT ( 'NONE',  ( 24.11042299814977952, -22.50654057154123677, -344.0834433819322840 ) ) ;
#48973=CARTESIAN_POINT ( 'NONE',  ( 172.5076325409972640, 241.1453524790508709, -177.1370813373998203 ) ) ;
#48975=CARTESIAN_POINT ( 'NONE',  ( 26.90366985021008261, -275.2273247194847272, -305.4689148819937827 ) ) ;
#48976=CARTESIAN_POINT ( 'NONE',  ( 26.91406211954589978, -273.9912076777142147, -234.9647298189462674 ) ) ;
#48977=CARTESIAN_POINT ( 'NONE',  ( -36.53512604192584945, -297.5696527736715211, -193.4227212417192732 ) ) ;
#48978=CARTESIAN_POINT ( 'NONE',  ( -106.9971877404514089, -265.1276182340686205, -305.5655013973570817 ) ) ;
#48979=CARTESIAN_POINT ( 'NONE',  ( 32.56234815641699498, -274.6363849193725173, -301.4532762367821874 ) ) ;
#48980=CARTESIAN_POINT ( 'NONE',  ( -60.93047101697215595, -299.6032995918266693, -199.9189876645664299 ) ) ;
#48981=CARTESIAN_POINT ( 'NONE',  ( -86.14501698932035367, -292.4363451673487475, -215.5893768787423994 ) ) ;
#48982=ORIENTED_EDGE ( 'NONE', *, *, #7422, .F. ) ;
#48983=CARTESIAN_POINT ( 'NONE',  ( -60.08983448113527714, -298.7057179334694865, -196.9890344714140156 ) ) ;
#48984=CARTESIAN_POINT ( 'NONE',  ( -15.82754909324679282, -289.2586977555125145, -340.2361187236685396 ) ) ;
#48985=CARTESIAN_POINT ( 'NONE',  ( -114.2044050404693252, -297.3284836599280538, -272.4755725938329078 ) ) ;
#48986=CARTESIAN_POINT ( 'NONE',  ( -33.43168903299599748, -295.4965446677736054, -347.2132710480843798 ) ) ;
#48987=CARTESIAN_POINT ( 'NONE',  ( 35.53452752329296516, -293.6522563999161548, -265.3142274651738717 ) ) ;
#48989=CARTESIAN_POINT ( 'NONE',  ( 38.18523616417426325, -277.5180562508114690, -273.9507054344690005 ) ) ;
#48991=CARTESIAN_POINT ( 'NONE',  ( -2.412472829965490728, -280.0093825389647577, -201.7936774572754928 ) ) ;
#48994=CARTESIAN_POINT ( 'NONE',  ( -91.13255127911651243, -278.7812074471644337, -320.1334881098632081 ) ) ;
#48995=CARTESIAN_POINT ( 'NONE',  ( 34.76120917754666095, -277.0044672212106320, -246.2132351918195070 ) ) ;
#48996=CARTESIAN_POINT ( 'NONE',  ( -51.03892439605401421, -275.2464802822533443, -344.4610022425868010 ) ) ;
#48997=CARTESIAN_POINT ( 'NONE',  ( -47.29482503177550967, -298.5738962064230577, -197.8886506911530603 ) ) ;
#48998=CARTESIAN_POINT ( 'NONE',  ( -108.5442712301038739, -294.8828204433801830, -289.0004685252769150 ) ) ;
#49000=CARTESIAN_POINT ( 'NONE',  ( -72.48430026534484227, -280.0919815571037361, -201.9028911782505986 ) ) ;
#49002=CARTESIAN_POINT ( 'NONE',  ( 19.18294190099698326, -276.3731083802287571, -316.5756738829676351 ) ) ;
#49004=CARTESIAN_POINT ( 'NONE',  ( 34.39766258241920127, -285.8987117250308074, -243.7761201490658891 ) ) ;
#49005=CARTESIAN_POINT ( 'NONE',  ( -9.970657782087727128, -300.3941834529350103, -195.1851368233604092 ) ) ;
#49007=AXIS2_PLACEMENT_3D ( 'NONE', #56861, #13293, #473 ) ;
#49008=CARTESIAN_POINT ( 'NONE',  ( 35.11888246362659061, -286.8834932232098254, -280.5549972923389532 ) ) ;
#49010=CARTESIAN_POINT ( 'NONE',  ( -68.93579284816676989, -277.8707398123788721, -203.4299046234843615 ) ) ;
#49011=CARTESIAN_POINT ( 'NONE',  ( -91.72008948157430552, -277.8322080479310330, -220.7792090945039831 ) ) ;
#49012=CARTESIAN_POINT ( 'NONE',  ( -93.66437921015022994, -281.9517676457292055, -319.0536172771480210 ) ) ;
#49013=CARTESIAN_POINT ( 'NONE',  ( 27.73743617622592339, -289.0538613437115600, -232.9797186796481583 ) ) ;
#49014=CARTESIAN_POINT ( 'NONE',  ( 27.12280758407763770, -277.2349098643475713, -305.5595377799446624 ) ) ;
#49016=CARTESIAN_POINT ( 'NONE',  ( -94.16280059709950478, -293.2310980993468661, -221.3888169776338373 ) ) ;
#49018=CARTESIAN_POINT ( 'NONE',  ( -69.88761212159255365, -275.7146826772521990, -339.0393140790539519 ) ) ;
#49019=CARTESIAN_POINT ( 'NONE',  ( -16.34366499675604700, -277.4250170473829940, -340.4354509730983978 ) ) ;
#49020=CARTESIAN_POINT ( 'NONE',  ( 37.45652204134463403, -283.6540100234881834, -278.2989887279164805 ) ) ;
#49022=CARTESIAN_POINT ( 'NONE',  ( 2.443119307038749355, -290.4439577755627511, -334.6602095165745254 ) ) ;
#49023=CARTESIAN_POINT ( 'NONE',  ( -110.6984052826173297, -294.7532517441525215, -254.6867332384633471 ) ) ;
#49026=CARTESIAN_POINT ( 'NONE',  ( 27.07680156465469423, -273.7557429711135910, -234.8784612666853491 ) ) ;
#49027=CARTESIAN_POINT ( 'NONE',  ( 21.17088218009146416, -291.0583096145643367, -224.6552685211873666 ) ) ;
#49030=CARTESIAN_POINT ( 'NONE',  ( -111.6377407753095525, -289.2516488475491201, -252.9597933251780262 ) ) ;
#49031=CARTESIAN_POINT ( 'NONE',  ( 38.34747920006685007, -285.6996990605342717, -263.0769924213881836 ) ) ;
#49032=CARTESIAN_POINT ( 'NONE',  ( -96.24842740309239275, -286.5915563871333802, -226.2547420232250204 ) ) ;
#49033=CARTESIAN_POINT ( 'NONE',  ( -14.52533024915295812, -287.1583125684668971, -200.7952885247583481 ) ) ;
#49034=CARTESIAN_POINT ( 'NONE',  ( -28.07686869166656507, -294.1489522567524091, -195.5251062565476161 ) ) ;
#49035=CARTESIAN_POINT ( 'NONE',  ( 36.49322979734465378, -273.8373710457436800, -286.4750576180215944 ) ) ;
#49036=CARTESIAN_POINT ( 'NONE',  ( 37.21932293740722031, -276.1250436357899503, -289.5026469455282268 ) ) ;
#49037=CARTESIAN_POINT ( 'NONE',  ( -112.6788521215020893, -288.5498593662401845, -276.8059660775163593 ) ) ;
#49038=CARTESIAN_POINT ( 'NONE',  ( -38.54495906529282223, -277.0668494516912688, -347.3517159015918310 ) ) ;
#49039=CARTESIAN_POINT ( 'NONE',  ( -87.57875334261140665, -297.7375328000662762, -325.5705853282494786 ) ) ;
#49041=CARTESIAN_POINT ( 'NONE',  ( 104.1717476309105166, -299.5541904835127980, -195.3611179825600175 ) ) ;
#49042=CARTESIAN_POINT ( 'NONE',  ( -110.3647210718829257, -283.1224591420339607, -279.1004827411406382 ) ) ;
#49043=CARTESIAN_POINT ( 'NONE',  ( -35.36259463782438672, -278.0768060983852479, -195.3744352578095231 ) ) ;
#49045=CARTESIAN_POINT ( 'NONE',  ( -24.25926044836468876, -272.6960145150854373, -195.1305954621356591 ) ) ;
#49046=CARTESIAN_POINT ( 'NONE',  ( -107.2165108551313892, -277.6145896345292385, -292.0109915301164847 ) ) ;
#49047=CARTESIAN_POINT ( 'NONE',  ( 34.74984846340299782, -295.2727566628387308, -285.7029626960218707 ) ) ;
#49048=CARTESIAN_POINT ( 'NONE',  ( 8.373349113323561355, -279.5815387699674375, -208.7189098049069855 ) ) ;
#49049=CARTESIAN_POINT ( 'NONE',  ( -28.85685618759001514, -295.8833435298444101, -343.1544157019758359 ) ) ;
#49050=CARTESIAN_POINT ( 'NONE',  ( -104.1639674885520606, -297.3799489035009174, -307.7263616356498801 ) ) ;
#49051=CARTESIAN_POINT ( 'NONE',  ( -55.29160844359187621, -297.6481932416154450, -199.5500571444789273 ) ) ;
#49052=CARTESIAN_POINT ( 'NONE',  ( -68.65891597376128175, -293.6407473882142085, -202.1983976820689008 ) ) ;
#49053=CARTESIAN_POINT ( 'NONE',  ( -52.17536325414393872, -286.0341051792089502, -194.7490513125552809 ) ) ;
#49054=CARTESIAN_POINT ( 'NONE',  ( 22.66923194685100640, -273.0642493935716857, -224.0907385376136176 ) ) ;
#49055=CARTESIAN_POINT ( 'NONE',  ( 19.62281679186269301, -288.0897526907239694, -322.1885150379844731 ) ) ;
#49056=CARTESIAN_POINT ( 'NONE',  ( -66.74020650577232061, -281.6450052654294609, -201.7354018456952645 ) ) ;
#49057=CARTESIAN_POINT ( 'NONE',  ( -4.478264524893772247, -285.5550389460045153, -204.9134056527796872 ) ) ;
#49058=CARTESIAN_POINT ( 'NONE',  ( -95.74903386913437942, -287.9043026848621594, -317.4301200119467126 ) ) ;
#49059=CARTESIAN_POINT ( 'NONE',  ( -84.42323508662160236, -232.9070939334762329, -346.4289530206739300 ) ) ;
#49060=CARTESIAN_POINT ( 'NONE',  ( 22.04526140838169113, -286.4644555410820885, -227.7178849848838240 ) ) ;
#49062=CARTESIAN_POINT ( 'NONE',  ( 25.74382143705825499, -283.0732098265501691, -314.1225217863477042 ) ) ;
#49063=CARTESIAN_POINT ( 'NONE',  ( -113.9522589089158799, -289.6718988075677430, -265.4987630313674458 ) ) ;
#49064=CARTESIAN_POINT ( 'NONE',  ( -92.50879621959956012, -280.8791148359696876, -217.7211551997537242 ) ) ;
#49065=CARTESIAN_POINT ( 'NONE',  ( -72.29653378419736498, -280.9146753078727556, -202.2917439333185428 ) ) ;
#49066=CARTESIAN_POINT ( 'NONE',  ( 19.35069529618707662, -282.0363800091801068, -316.3696488228370072 ) ) ;
#49067=CARTESIAN_POINT ( 'NONE',  ( 35.18251157533608620, -277.7979341069139423, -289.4723546865220669 ) ) ;
#49068=CARTESIAN_POINT ( 'NONE',  ( -5.797701210098003877, -294.6487355951004474, -340.6033854022714991 ) ) ;
#49069=CARTESIAN_POINT ( 'NONE',  ( -101.7353558642199829, -288.0641249232600671, -308.2161762152076676 ) ) ;
#49070=CARTESIAN_POINT ( 'NONE',  ( -94.19094351354441130, -294.8198855719933249, -316.6668060364984285 ) ) ;
#49072=CARTESIAN_POINT ( 'NONE',  ( -69.61171599948387723, -285.4004398315260005, -337.4569337373252438 ) ) ;
#49073=CARTESIAN_POINT ( 'NONE',  ( -73.31651649521867853, -295.2101576183756606, -333.9055911816712978 ) ) ;
#49074=CARTESIAN_POINT ( 'NONE',  ( -7.323915927691939665, -293.5163528241192239, -199.7747278483543880 ) ) ;
#49076=CARTESIAN_POINT ( 'NONE',  ( -40.23009277398153216, -283.7408306292705333, -343.4059662359040317 ) ) ;
#49077=CARTESIAN_POINT ( 'NONE',  ( -35.51732685292294178, -273.1332410854584509, -193.6050031194094743 ) ) ;
#49078=CARTESIAN_POINT ( 'NONE',  ( -40.63636649869368966, -292.6631778737889249, -193.5204975093755024 ) ) ;
#49079=CARTESIAN_POINT ( 'NONE',  ( -80.21933912314375448, -283.6183068140346109, -207.8333060438608868 ) ) ;
#49080=CARTESIAN_POINT ( 'NONE',  ( -104.5935665005996924, -291.3711356347590140, -232.9054006504900940 ) ) ;
#49081=CARTESIAN_POINT ( 'NONE',  ( -5.779451788039407845, -288.9585810550704537, -336.2087600557789528 ) ) ;
#49085=CARTESIAN_POINT ( 'NONE',  ( 102.9770308486741328, 114.5320353338112795, -279.4838030456201068 ) ) ;
#49086=CARTESIAN_POINT ( 'NONE',  ( 15.28944551476376645, -283.8448576489772677, -325.6120931757356516 ) ) ;
#49087=CARTESIAN_POINT ( 'NONE',  ( -54.42813229853333468, -289.3380690714489560, -195.3538533559490702 ) ) ;
#49089=CARTESIAN_POINT ( 'NONE',  ( 22.05434560458958870, -281.0713194943489270, -313.3516161058334433 ) ) ;
#49090=CARTESIAN_POINT ( 'NONE',  ( -45.65155453694142551, -276.8213249183204994, -346.9431800961029921 ) ) ;
#49091=CARTESIAN_POINT ( 'NONE',  ( -90.36735601340649282, -279.8044037143159812, -323.2391095640879826 ) ) ;
#49092=CARTESIAN_POINT ( 'NONE',  ( 140.4625507534157975, 178.1663472580048335, -239.4196196848511420 ) ) ;
#49093=CARTESIAN_POINT ( 'NONE',  ( 14.77283351634792119, -279.3435719254887317, -214.4078117668306618 ) ) ;
#49094=CARTESIAN_POINT ( 'NONE',  ( -65.69514492888039570, -283.6997393491515709, -201.2559156838794365 ) ) ;
#49095=CARTESIAN_POINT ( 'NONE',  ( -111.6148598902819060, -298.5163616957030968, -254.2543746898427912 ) ) ;
#49097=CARTESIAN_POINT ( 'NONE',  ( 31.85729972201680482, -293.7314282135134249, -246.7625333284971418 ) ) ;
#49099=CARTESIAN_POINT ( 'NONE',  ( -109.4256946558087549, -289.0484576283844262, -284.7483117707091083 ) ) ;
#49100=CARTESIAN_POINT ( 'NONE',  ( 39.60548046197511951, -276.2135972914053355, -271.1622903833703617 ) ) ;
#49101=CARTESIAN_POINT ( 'NONE',  ( -97.84319116648059378, -273.1209974988395288, -229.4228094201411352 ) ) ;
#49103=CARTESIAN_POINT ( 'NONE',  ( 120.8395553409046528, -299.5541904835127980, -192.4214616598467273 ) ) ;
#49107=CARTESIAN_POINT ( 'NONE',  ( 35.44840891232407643, -282.7516556034379960, -279.4831145160931669 ) ) ;
#49108=CARTESIAN_POINT ( 'NONE',  ( -69.55347985637641273, -281.3941751992882701, -201.5255879351402655 ) ) ;
#49109=CARTESIAN_POINT ( 'NONE',  ( -48.37592472953704004, -282.2547953711271589, -342.7603882486318412 ) ) ;
#49110=CARTESIAN_POINT ( 'NONE',  ( 36.93908527581412216, -283.4248356664701873, -271.3062335397923448 ) ) ;
#49111=CARTESIAN_POINT ( 'NONE',  ( 20.55527005517390293, -274.6693526733768067, -315.9736327882210389 ) ) ;
#49114=CARTESIAN_POINT ( 'NONE',  ( -100.3272692630247604, -278.7719550302677476, -314.3722177343089470 ) ) ;
#49115=VERTEX_POINT ( 'NONE', #87206 ) ;
#49118=CARTESIAN_POINT ( 'NONE',  ( -93.16339709568981675, -285.8291524398680963, -320.9998585473391017 ) ) ;
#49119=CARTESIAN_POINT ( 'NONE',  ( 18.08809796983242535, -293.4280714735289166, -318.1310194508695872 ) ) ;
#49121=CARTESIAN_POINT ( 'NONE',  ( 35.84818837399613045, -287.1978113967840613, -293.9524936863486460 ) ) ;
#49122=CARTESIAN_POINT ( 'NONE',  ( -16.87038407043041843, -284.5598833568400323, -199.1815926201236095 ) ) ;
#49123=CARTESIAN_POINT ( 'NONE',  ( -97.83000789474490944, -283.7064039238655369, -228.4277605393226054 ) ) ;
#49124=CARTESIAN_POINT ( 'NONE',  ( 21.97231311791058062, -286.4049401136632014, -314.6522005231041135 ) ) ;
#49125=CARTESIAN_POINT ( 'NONE',  ( 22.14270585578276140, -283.3556974694646442, -313.3795724948092243 ) ) ;
#49126=CARTESIAN_POINT ( 'NONE',  ( 21.21329987222718216, -272.9073229016873938, -223.4759093354347215 ) ) ;
#49127=CARTESIAN_POINT ( 'NONE',  ( -37.95534399401411463, -284.4444628814347880, -194.1635861345968976 ) ) ;
#49128=CARTESIAN_POINT ( 'NONE',  ( -67.39993049667045000, -299.6582395602201814, -201.5925882785752776 ) ) ;
#49129=CARTESIAN_POINT ( 'NONE',  ( -106.2353503082650406, -282.9460941968366114, -240.1695816952180564 ) ) ;
#49130=CARTESIAN_POINT ( 'NONE',  ( -19.48876145229224477, -281.2285886096219656, -199.2827438418755150 ) ) ;
#49131=CARTESIAN_POINT ( 'NONE',  ( 21.53947659948623539, -288.9115637224510351, -223.6176472908123571 ) ) ;
#49134=CARTESIAN_POINT ( 'NONE',  ( -8.906817434781190812, -296.6034004334743486, -340.4220638305647526 ) ) ;
#49135=CARTESIAN_POINT ( 'NONE',  ( -111.5983994372167274, -276.6918485240350947, -259.4686532257498470 ) ) ;
#49136=CARTESIAN_POINT ( 'NONE',  ( -96.27380454153264111, -289.0841801484867233, -319.6883841592798490 ) ) ;
#49137=CARTESIAN_POINT ( 'NONE',  ( -31.55978762442567032, -293.3779524982520002, -343.9849407873743417 ) ) ;
#49138=CARTESIAN_POINT ( 'NONE',  ( -4.109692083600355872, -279.1846349974526902, -204.7965626360831095 ) ) ;
#49139=CARTESIAN_POINT ( 'NONE',  ( -90.24877788817013879, -271.3763951383644439, -217.9955250806533229 ) ) ;
#49140=CARTESIAN_POINT ( 'NONE',  ( 34.42778658241596190, -294.6592285785947638, -254.4794508867490492 ) ) ;
#49141=CARTESIAN_POINT ( 'NONE',  ( -85.33152481854862970, -287.9090924074130839, -210.2361428286348826 ) ) ;
#49142=CARTESIAN_POINT ( 'NONE',  ( -110.9285790518850519, -294.7768201939189794, -290.5521804639286643 ) ) ;
#49143=CARTESIAN_POINT ( 'NONE',  ( 16.60957983065679500, -289.8693134514361986, -320.7916479551012685 ) ) ;
#49144=CARTESIAN_POINT ( 'NONE',  ( -6.280375931710404203, -290.6944730099417598, -200.9988491171323517 ) ) ;
#49146=CARTESIAN_POINT ( 'NONE',  ( -97.02596226968955762, -291.3801880719717019, -313.4095066944574910 ) ) ;
#49148=CARTESIAN_POINT ( 'NONE',  ( -72.71396675743028482, -292.3741618894063095, -206.2619765764734154 ) ) ;
#49149=CARTESIAN_POINT ( 'NONE',  ( 104.2209783822911646, -299.5541904835127980, -195.3611179825600175 ) ) ;
#49150=CARTESIAN_POINT ( 'NONE',  ( -107.3621537013787162, -291.3572299554362530, -301.5583013647922712 ) ) ;
#49151=CARTESIAN_POINT ( 'NONE',  ( 30.89209248614742975, -279.9920850561903194, -302.4614010193409968 ) ) ;
#49152=CARTESIAN_POINT ( 'NONE',  ( -0.09095052937821483663, -292.5628401401612564, -207.5806938494377505 ) ) ;
#49153=CARTESIAN_POINT ( 'NONE',  ( 23.74730553436537051, -280.9266612193979427, -223.4659889627629070 ) ) ;
#49154=CARTESIAN_POINT ( 'NONE',  ( -111.4722552536914293, -283.9588377413188027, -291.1073245836867613 ) ) ;
#49156=CARTESIAN_POINT ( 'NONE',  ( -75.67640438035840589, -287.5647585583109844, -334.6449780943910923 ) ) ;
#49157=CARTESIAN_POINT ( 'NONE',  ( 23.13327050988670308, -279.1003461945784352, -227.3071587224978600 ) ) ;
#49158=CARTESIAN_POINT ( 'NONE',  ( -70.16728794738936870, -283.6194677676351148, -202.9261015755886888 ) ) ;
#49160=CARTESIAN_POINT ( 'NONE',  ( -9.099565082630544310, -278.8947312874761337, -199.4732518768447562 ) ) ;
#49162=CARTESIAN_POINT ( 'NONE',  ( 34.56917776149460764, -286.1341763958552633, -243.7093234773917061 ) ) ;
#49164=CARTESIAN_POINT ( 'NONE',  ( 29.45401654481353759, -294.7315408916153388, -238.8594921247345439 ) ) ;
#49165=CARTESIAN_POINT ( 'NONE',  ( 23.15512436067898250, -276.3494060077114796, -223.6628461444487073 ) ) ;
#49166=CARTESIAN_POINT ( 'NONE',  ( -109.5136063674918603, -278.0724289027510849, -281.4653260391751814 ) ) ;
#49167=CARTESIAN_POINT ( 'NONE',  ( -98.34956489679777292, -291.3459372703922554, -223.3606332760649025 ) ) ;
#49168=CARTESIAN_POINT ( 'NONE',  ( -96.06894653456953392, -281.9820175020212218, -317.9253823626308417 ) ) ;
#49169=CARTESIAN_POINT ( 'NONE',  ( -110.4798827387940747, -289.6720697204048633, -265.7087646233287614 ) ) ;
#49170=CARTESIAN_POINT ( 'NONE',  ( -71.19469432189183067, -293.4989171445441229, -337.2862659958021823 ) ) ;
#49173=CARTESIAN_POINT ( 'NONE',  ( -38.89260454416110946, -291.5398259189723831, -197.3160419175862899 ) ) ;
#49174=CARTESIAN_POINT ( 'NONE',  ( -102.0172624299487154, -276.4809262143062369, -239.1787733560258289 ) ) ;
#49175=CARTESIAN_POINT ( 'NONE',  ( -97.15544886054213691, -296.2577419959949907, -222.2452611705070353 ) ) ;
#49176=CARTESIAN_POINT ( 'NONE',  ( 28.67382479035883591, -280.1832238765678085, -307.6466859644883129 ) ) ;
#49177=CARTESIAN_POINT ( 'NONE',  ( -107.7665951037462264, -285.4828190352072852, -300.3902620803494301 ) ) ;
#49178=CARTESIAN_POINT ( 'NONE',  ( 32.27423283835092604, -287.0937559301826809, -248.3506084061936861 ) ) ;
#49179=CARTESIAN_POINT ( 'NONE',  ( 20.57931060041919125, -277.7091043712395049, -315.9430999488069460 ) ) ;
#49180=CARTESIAN_POINT ( 'NONE',  ( -69.24267329968802187, -293.4939513421193737, -337.8597861783933354 ) ) ;
#49181=CARTESIAN_POINT ( 'NONE',  ( -70.15342174942310294, -297.2507374106174325, -336.7039016190236680 ) ) ;
#49182=CARTESIAN_POINT ( 'NONE',  ( -18.93208968318285201, -275.6047359527323692, -341.4119219677253341 ) ) ;
#49183=ORIENTED_EDGE ( 'NONE', *, *, #85799, .T. ) ;
#49185=CARTESIAN_POINT ( 'NONE',  ( -84.17570399533069292, -295.3427602249360575, -331.5210473798308044 ) ) ;
#49186=CARTESIAN_POINT ( 'NONE',  ( 28.31181303545864836, -289.9425791577672271, -305.5555103011849383 ) ) ;
#49187=CARTESIAN_POINT ( 'NONE',  ( -35.71110069026453004, -296.0724073071932594, -195.3616651891954064 ) ) ;
#49188=CARTESIAN_POINT ( 'NONE',  ( -8.170200181195644618, -289.3112761448499555, -337.4444557185789790 ) ) ;
#49189=ORIENTED_EDGE ( 'NONE', *, *, #61048, .T. ) ;
#49190=CARTESIAN_POINT ( 'NONE',  ( -7.616997862642444161, -279.4911197246729557, -199.5707153718254858 ) ) ;
#49191=CARTESIAN_POINT ( 'NONE',  ( -88.53138469905071872, -296.3990029082412434, -327.8165643881372944 ) ) ;
#49192=CARTESIAN_POINT ( 'NONE',  ( -111.0663494786645629, -288.4690682680628697, -287.8804222091131919 ) ) ;
#49193=CARTESIAN_POINT ( 'NONE',  ( -74.59240837974009253, -295.8667219565606956, -337.7864496464563899 ) ) ;
#49194=CARTESIAN_POINT ( 'NONE',  ( 33.13822410391224338, -294.1381844362985589, -289.5049464147945173 ) ) ;
#49198=CARTESIAN_POINT ( 'NONE',  ( 31.07444624205723827, -289.5118094743826305, -304.2729300940271742 ) ) ;
#49199=CARTESIAN_POINT ( 'NONE',  ( 40.65961533371913106, -278.2662352645559167, -288.1317622949166548 ) ) ;
#49200=CARTESIAN_POINT ( 'NONE',  ( 31.93324942420514745, -280.4705606480367237, -236.8575417386156516 ) ) ;
#49201=CARTESIAN_POINT ( 'NONE',  ( 2.088426583040009277, -284.5235453671684240, -334.0242595690198755 ) ) ;
#49202=CARTESIAN_POINT ( 'NONE',  ( 21.64695662328472991, -285.4693332063245066, -221.7921498064391699 ) ) ;
#49203=CARTESIAN_POINT ( 'NONE',  ( -98.54655273510253721, -288.0528547896117288, -312.7542694945253743 ) ) ;
#49204=CARTESIAN_POINT ( 'NONE',  ( -7.046488210190877233, -278.5193210699403608, -339.8194104634520727 ) ) ;
#49205=ORIENTED_EDGE ( 'NONE', *, *, #18309, .F. ) ;
#49206=CARTESIAN_POINT ( 'NONE',  ( -107.1166226041311376, -278.2658977376094640, -291.9887221695387893 ) ) ;
#49207=CARTESIAN_POINT ( 'NONE',  ( -22.16515713726739634, -279.6001634413627812, -198.7999905016983462 ) ) ;
#49208=CARTESIAN_POINT ( 'NONE',  ( -35.70426938834810926, -278.1117608034664386, -347.0475956436979459 ) ) ;
#49209=CARTESIAN_POINT ( 'NONE',  ( -111.0625828863430797, -277.0848660179694889, -291.1755400136414664 ) ) ;
#49210=CARTESIAN_POINT ( 'NONE',  ( -40.88237375196717949, -139.0235881544214465, -362.1721031521604459 ) ) ;
#49211=CARTESIAN_POINT ( 'NONE',  ( -90.01016813982198528, -274.2713533787037363, -214.4418274450818274 ) ) ;
#49213=CARTESIAN_POINT ( 'NONE',  ( -37.27248207896832355, -299.4782701078396485, -193.9495680680081193 ) ) ;
#49215=CARTESIAN_POINT ( 'NONE',  ( -54.49178911615187815, -282.3376638359844719, -195.3683826091709363 ) ) ;
#49218=CARTESIAN_POINT ( 'NONE',  ( 20.57645075312527183, -288.0014731788448898, -225.4198911066196445 ) ) ;
#49219=CARTESIAN_POINT ( 'NONE',  ( -43.60538776689624285, -287.7343192976260298, -194.5804915227278400 ) ) ;
#49220=CARTESIAN_POINT ( 'NONE',  ( -29.16995199311165265, -288.2944427489298391, -343.0048733955921421 ) ) ;
#49221=CARTESIAN_POINT ( 'NONE',  ( -81.53134274645626078, -283.1430784093630564, -333.4084919218286700 ) ) ;
#49222=CARTESIAN_POINT ( 'NONE',  ( 11.85410503779443125, -279.1492084297348129, -215.3500902929334302 ) ) ;
#49223=CARTESIAN_POINT ( 'NONE',  ( -10.32210001801530375, -288.2689450926400241, -201.2039874693329864 ) ) ;
#49224=CARTESIAN_POINT ( 'NONE',  ( -4.016879618372591665, -278.9797202015645325, -204.6191383521114915 ) ) ;
#49225=CARTESIAN_POINT ( 'NONE',  ( -7.290784495181046765, -277.9647077617255491, -337.4296348058483659 ) ) ;
#49226=CARTESIAN_POINT ( 'NONE',  ( -85.14077061281625447, -278.2252856588017949, -325.6842358528556360 ) ) ;
#49227=CARTESIAN_POINT ( 'NONE',  ( 25.51704155755779624, -286.9297003222523585, -314.2332990256165317 ) ) ;
#49229=CARTESIAN_POINT ( 'NONE',  ( -47.22544400801635334, -283.9775268795589227, -346.5613176351404832 ) ) ;
#49230=CARTESIAN_POINT ( 'NONE',  ( -101.3644475367764954, -284.4813648353229496, -313.1253625659184650 ) ) ;
#49231=CARTESIAN_POINT ( 'NONE',  ( 28.97179329763490330, -281.3056288400366611, -239.7191616712284485 ) ) ;
#49235=CARTESIAN_POINT ( 'NONE',  ( -111.1199614985169575, -292.6316394586439174, -253.1252938378680710 ) ) ;
#49236=CARTESIAN_POINT ( 'NONE',  ( -36.36771406311004995, -290.7489564975377903, -193.8475175711297425 ) ) ;
#49237=CARTESIAN_POINT ( 'NONE',  ( -105.6313159127634691, -271.9649432963055915, -243.7649708839908556 ) ) ;
#49239=CARTESIAN_POINT ( 'NONE',  ( -3.281404455394420605, -293.9628268995140843, -339.3192226677529675 ) ) ;
#49240=CARTESIAN_POINT ( 'NONE',  ( -107.6191108771980254, -288.7388302356640111, -292.7064533077071928 ) ) ;
#49241=CARTESIAN_POINT ( 'NONE',  ( 33.71685718705287371, -292.0626699972600591, -291.1106181194548412 ) ) ;
#49242=CARTESIAN_POINT ( 'NONE',  ( -21.02622964997116028, -290.0431767370299099, -341.9218329502278380 ) ) ;
#49243=CARTESIAN_POINT ( 'NONE',  ( 99.44099354567467230, -302.2645883696979467, -195.3030568020281521 ) ) ;
#49244=CARTESIAN_POINT ( 'NONE',  ( -77.05520120966228603, -291.5840230157716633, -334.0443139884949915 ) ) ;
#49245=CARTESIAN_POINT ( 'NONE',  ( -89.49512086895755658, -289.3196994208087744, -216.1589757877136435 ) ) ;
#49246=CARTESIAN_POINT ( 'NONE',  ( -100.2445566975779059, -293.1040255495365727, -229.4241609441090475 ) ) ;
#49247=CARTESIAN_POINT ( 'NONE',  ( -19.77097385643332217, -287.2249183327063520, -199.2648591100277145 ) ) ;
#49248=CARTESIAN_POINT ( 'NONE',  ( 37.77570333207331288, -295.5871765842871355, -273.0821694437856877 ) ) ;
#49249=CARTESIAN_POINT ( 'NONE',  ( -114.3482646169705674, -272.5982171866134536, -270.3617045005363480 ) ) ;
#49251=CARTESIAN_POINT ( 'NONE',  ( 8.489571720350356898, -276.6562200302269048, -210.5455571263578634 ) ) ;
#49252=CARTESIAN_POINT ( 'NONE',  ( -86.30030961089215680, -294.9091377980266770, -329.5828486015593626 ) ) ;
#49253=CARTESIAN_POINT ( 'NONE',  ( -32.60408444673965533, -272.3525055224150719, -196.4868649115544770 ) ) ;
#49254=CARTESIAN_POINT ( 'NONE',  ( -98.85223252442033015, -276.0600179606722691, -312.2868690514748664 ) ) ;
#49255=CARTESIAN_POINT ( 'NONE',  ( 95.51333995075087557, -301.0646807905992546, -196.8375845645956588 ) ) ;
#49256=CARTESIAN_POINT ( 'NONE',  ( -13.23107632313859661, -272.9340728762614958, -197.8539865288538238 ) ) ;
#49258=CARTESIAN_POINT ( 'NONE',  ( -104.4666997236304127, -297.5729298646509733, -300.6453423370959399 ) ) ;
#49260=CARTESIAN_POINT ( 'NONE',  ( -108.6366949056745739, -297.5711199410398535, -253.9408424904898709 ) ) ;
#49261=CARTESIAN_POINT ( 'NONE',  ( 11.04123961856805991, -284.7376718077125020, -212.5219273896025811 ) ) ;
#49262=CARTESIAN_POINT ( 'NONE',  ( -41.86834226397009928, -297.9935230211907538, -197.5015989684078477 ) ) ;
#49263=CARTESIAN_POINT ( 'NONE',  ( -3.489356550369109744, -286.4866871607825942, -201.1872173472987697 ) ) ;
#49264=CARTESIAN_POINT ( 'NONE',  ( -65.44326090546300634, -289.0762355400047454, -342.0836633563843634 ) ) ;
#49265=CARTESIAN_POINT ( 'NONE',  ( -98.59949036658522914, -299.1262371542309779, -226.4761554149631024 ) ) ;
#49266=CARTESIAN_POINT ( 'NONE',  ( 4.829037383091367985, -292.4808522074100665, -332.1806725105772102 ) ) ;
#49267=CARTESIAN_POINT ( 'NONE',  ( -6.286237524601067328, -279.6470145315262243, -200.0637538910139881 ) ) ;
#49268=CARTESIAN_POINT ( 'NONE',  ( -85.28047601435908120, -282.9094976428775681, -210.1954327657594206 ) ) ;
#49270=CARTESIAN_POINT ( 'NONE',  ( 26.03118902092522546, -286.8537637568193190, -307.4886777664013948 ) ) ;
#49272=CARTESIAN_POINT ( 'NONE',  ( -100.5404131816323030, -288.0083156826877371, -310.7458095915461058 ) ) ;
#49273=CARTESIAN_POINT ( 'NONE',  ( 96.20670667332062465, -301.3513922989450293, -196.5240784471901634 ) ) ;
#49274=CARTESIAN_POINT ( 'NONE',  ( -64.54962249166925403, -281.1292334848691894, -198.9026848043201312 ) ) ;
#49275=CARTESIAN_POINT ( 'NONE',  ( -109.2382278915457476, -294.2820011147274499, -292.9719442165803684 ) ) ;
#49276=CARTESIAN_POINT ( 'NONE',  ( 13.92468116014686963, -282.3085731703355350, -322.4011092763580564 ) ) ;
#49277=CARTESIAN_POINT ( 'NONE',  ( -114.1209986064743305, -296.7999800278627731, -263.8725706023754469 ) ) ;
#49278=CARTESIAN_POINT ( 'NONE',  ( -94.24548768623192530, -274.6332888950271354, -223.6794988190263496 ) ) ;
#49279=CARTESIAN_POINT ( 'NONE',  ( 37.29067828820828367, -283.6540100242638687, -278.2813320565020376 ) ) ;
#49280=CARTESIAN_POINT ( 'NONE',  ( -110.0395646704508437, -295.4890986399194617, -279.6237507618450877 ) ) ;
#49282=CARTESIAN_POINT ( 'NONE',  ( -21.00420178891176093, -284.8215222325350737, -343.2492770160816917 ) ) ;
#49284=CARTESIAN_POINT ( 'NONE',  ( -37.37352853689063181, -286.5523547857347353, -345.3611179825600175 ) ) ;
#49285=CARTESIAN_POINT ( 'NONE',  ( -22.97913104049548849, -276.0702068303619399, -345.8994609378297014 ) ) ;
#49286=CARTESIAN_POINT ( 'NONE',  ( -33.50631320998932949, -291.9350573156178825, -197.4494501609347310 ) ) ;
#49287=CARTESIAN_POINT ( 'NONE',  ( 16.34411708659709461, -283.7928447098638571, -320.9178358879467510 ) ) ;
#49289=CARTESIAN_POINT ( 'NONE',  ( 29.80556030941353640, -276.7424239733973650, -239.6159136246452590 ) ) ;
#49290=CARTESIAN_POINT ( 'NONE',  ( -113.0132238756227423, -285.8390894433941867, -281.3373609543272096 ) ) ;
#49291=CARTESIAN_POINT ( 'NONE',  ( -108.4818575970703876, -283.1099788768923986, -288.4223610517784664 ) ) ;
#49292=CARTESIAN_POINT ( 'NONE',  ( -110.4296838251088957, -280.3355224867646598, -287.2449320147026128 ) ) ;
#49293=CARTESIAN_POINT ( 'NONE',  ( -83.58178668456264404, -273.6044625959950736, -208.7244688315625183 ) ) ;
#49294=CARTESIAN_POINT ( 'NONE',  ( 16.95372047719630970, -276.1380398866648989, -325.0341703442957169 ) ) ;
#49295=CARTESIAN_POINT ( 'NONE',  ( 34.13966513139777703, -295.7423709774723193, -291.1850664419484360 ) ) ;
#49299=CARTESIAN_POINT ( 'NONE',  ( -105.3933162352427360, -295.1264214598473927, -237.0552172594741194 ) ) ;
#49300=CARTESIAN_POINT ( 'NONE',  ( 35.16635195036931805, -275.1834271174261630, -279.7404480648376648 ) ) ;
#49301=CARTESIAN_POINT ( 'NONE',  ( 3.869287891386177680, -296.0286083279678451, -334.6445354065239712 ) ) ;
#49302=CARTESIAN_POINT ( 'NONE',  ( -19.36549193832724569, -296.0310787375668724, -344.8795710410058177 ) ) ;
#49303=CARTESIAN_POINT ( 'NONE',  ( -99.84448409623446707, -293.1101111241127342, -229.1156338941977424 ) ) ;
#49305=CARTESIAN_POINT ( 'NONE',  ( -77.35715088523424754, -275.5895855800703771, -333.6580764922073854 ) ) ;
#49306=CARTESIAN_POINT ( 'NONE',  ( -109.2041406534285102, -280.2207571825831565, -289.7802796998409463 ) ) ;
#49307=CARTESIAN_POINT ( 'NONE',  ( -110.5629126595498093, -294.4575359338207363, -283.8470796261016176 ) ) ;
#49308=CARTESIAN_POINT ( 'NONE',  ( 38.29766792498102745, -283.4785496407121173, -275.5522773263807608 ) ) ;
#49309=CARTESIAN_POINT ( 'NONE',  ( -74.86657584358310658, -284.4600258705754072, -207.3840604443440441 ) ) ;
#49310=CARTESIAN_POINT ( 'NONE',  ( 199.0839727162727115, 283.4321579852195896, -111.4451161440015596 ) ) ;
#49312=CARTESIAN_POINT ( 'NONE',  ( -107.4134080596330847, -283.9466203996772151, -290.9494618193027691 ) ) ;
#49314=CARTESIAN_POINT ( 'NONE',  ( 39.31128206412358850, -282.6620961325044163, -272.7720990991858230 ) ) ;
#49315=CARTESIAN_POINT ( 'NONE',  ( -113.8130298055446303, -283.2802780066679134, -275.6748678080809896 ) ) ;
#49316=CARTESIAN_POINT ( 'NONE',  ( -103.3971930608186085, -278.9811672193897039, -309.5740526285790679 ) ) ;
#49317=CARTESIAN_POINT ( 'NONE',  ( -108.0070055901374673, -279.7032373881422700, -299.1556027865092915 ) ) ;
#49318=CARTESIAN_POINT ( 'NONE',  ( -14.26626197960825415, -280.9950113884769962, -196.9511055558885744 ) ) ;
#49319=CARTESIAN_POINT ( 'NONE',  ( -82.08285599513421005, -270.9094976428775681, -214.2051214447836571 ) ) ;
#49320=CARTESIAN_POINT ( 'NONE',  ( 104.0975919659984754, 115.9579523938436125, -282.9976511085191078 ) ) ;
#49323=CARTESIAN_POINT ( 'NONE',  ( 0.3558082256967267654, -276.5556580839059961, -205.7015479880308533 ) ) ;
#49324=CARTESIAN_POINT ( 'NONE',  ( 64.32927610681132080, 48.12963783785930616, -318.7087835613883726 ) ) ;
#49325=CARTESIAN_POINT ( 'NONE',  ( -6.057569129089722004, -278.4854132110050386, -202.5743814259453188 ) ) ;
#49326=CARTESIAN_POINT ( 'NONE',  ( 1.166968862343012558, -294.3186248787766885, -204.7948394867840420 ) ) ;
#49327=CARTESIAN_POINT ( 'NONE',  ( 17.15102308680967980, -293.5970225384867263, -319.1081707556673450 ) ) ;
#49328=CARTESIAN_POINT ( 'NONE',  ( -71.88446366406991217, -289.0041896723178070, -339.1093862574692253 ) ) ;
#49330=CARTESIAN_POINT ( 'NONE',  ( 8.537774792222245779, -293.0120981470960260, -331.4649646075354212 ) ) ;
#49331=CARTESIAN_POINT ( 'NONE',  ( -94.73143348198347269, -283.6013342620691446, -223.9421858382964956 ) ) ;
#49332=CARTESIAN_POINT ( 'NONE',  ( -106.8758198994898407, -292.7553319339965014, -244.2175961206301338 ) ) ;
#49333=CARTESIAN_POINT ( 'NONE',  ( 7.362744667237497431, -285.1537609073272392, -211.7114757675392127 ) ) ;
#49334=CARTESIAN_POINT ( 'NONE',  ( -108.8492087245877542, -286.0903214198768296, -253.3386690343470491 ) ) ;
#49336=CARTESIAN_POINT ( 'NONE',  ( -95.49054990725012715, -292.1723607676894403, -220.2258401223970736 ) ) ;
#49337=CARTESIAN_POINT ( 'NONE',  ( -13.50336789250761704, -283.2266078969134924, -339.4779459847818543 ) ) ;
#49338=CARTESIAN_POINT ( 'NONE',  ( -27.81252489032839748, -293.7287728309499357, -346.4220525941694291 ) ) ;
#49339=CARTESIAN_POINT ( 'NONE',  ( -26.15794092729106879, -289.7160529415188535, -346.3813938979574800 ) ) ;
#49340=CARTESIAN_POINT ( 'NONE',  ( -48.85359180828439918, -289.6872350485109564, -346.4873740311346637 ) ) ;
#49341=CARTESIAN_POINT ( 'NONE',  ( 26.36634333461551449, -287.2300712122791424, -234.6166380906255426 ) ) ;
#49344=CARTESIAN_POINT ( 'NONE',  ( -110.0236366759265962, -298.1393170590828277, -291.7993876164754283 ) ) ;
#49345=CARTESIAN_POINT ( 'NONE',  ( -100.3350459130212045, -295.8141725894475371, -226.9199416932148665 ) ) ;
#49346=CARTESIAN_POINT ( 'NONE',  ( -41.05115383850343136, -279.0630680189487975, -197.2198273069739116 ) ) ;
#49347=CARTESIAN_POINT ( 'NONE',  ( -96.88445487593706673, -272.7147279018413428, -221.6149287202791243 ) ) ;
#49348=CARTESIAN_POINT ( 'NONE',  ( -35.65396063747169109, -293.5105063549002011, -344.0477398844732306 ) ) ;
#49349=CARTESIAN_POINT ( 'NONE',  ( 24.84784978655136811, -277.8613295289777056, -310.5858722263483855 ) ) ;
#49350=CARTESIAN_POINT ( 'NONE',  ( -40.53962720997532898, -296.2512795178856777, -196.4041775417347822 ) ) ;
#49351=CARTESIAN_POINT ( 'NONE',  ( -63.69732051053190958, -296.6084910984629346, -338.9168728220820412 ) ) ;
#49352=CARTESIAN_POINT ( 'NONE',  ( -55.86820583086120706, -296.3758951696924555, -341.3432250714157021 ) ) ;
#49354=CARTESIAN_POINT ( 'NONE',  ( -70.44174824770956889, -297.0812530218202596, -339.0109421419915066 ) ) ;
#49355=CARTESIAN_POINT ( 'NONE',  ( -94.16796324185864364, -295.2335761247824735, -221.0817999478998672 ) ) ;
#49356=CARTESIAN_POINT ( 'NONE',  ( -60.29883678888856480, -292.3980457138673046, -200.9043809704727437 ) ) ;
#49357=CARTESIAN_POINT ( 'NONE',  ( 30.66798256948669987, -299.5341108523645062, -193.4557286876616047 ) ) ;
#49358=CARTESIAN_POINT ( 'NONE',  ( -94.57390594131445027, -288.4778583820977360, -316.6196257060797166 ) ) ;
#49359=CARTESIAN_POINT ( 'NONE',  ( -49.21654576272059245, -275.9011149203553259, -196.2545826088790193 ) ) ;
#49360=CARTESIAN_POINT ( 'NONE',  ( -31.27117788039909030, -274.6192046584260993, -193.6492445006108483 ) ) ;
#49361=CARTESIAN_POINT ( 'NONE',  ( -77.52715254868695638, -297.8300554375055640, -209.3313719314394064 ) ) ;
#49362=CARTESIAN_POINT ( 'NONE',  ( -58.85716409511214664, -281.7550661210618728, -198.1427573624997081 ) ) ;
#49363=CARTESIAN_POINT ( 'NONE',  ( -9.027948151839110480, -279.0996461557298289, -199.2863002059818314 ) ) ;
#49365=CARTESIAN_POINT ( 'NONE',  ( -35.90942285938511702, -282.3832550318252856, -347.2589454746797060 ) ) ;
#49366=CARTESIAN_POINT ( 'NONE',  ( 36.39335892120758587, -275.1754757295692571, -292.2353815850151477 ) ) ;
#49367=CARTESIAN_POINT ( 'NONE',  ( 38.61589809767567516, -279.8752741457325897, -264.2879239529505071 ) ) ;
#49368=CARTESIAN_POINT ( 'NONE',  ( 37.36374049901815653, -279.4396171921135874, -261.5898087648716910 ) ) ;
#49370=CARTESIAN_POINT ( 'NONE',  ( -38.07012738008141639, -272.6175739945053920, -196.7754922617695570 ) ) ;
#49371=CARTESIAN_POINT ( 'NONE',  ( -106.8900582768564789, -280.1848723049914156, -298.5698349694508806 ) ) ;
#49373=PLANE ( 'NONE',  #23252 ) ;
#49374=CARTESIAN_POINT ( 'NONE',  ( -51.58835398563933694, -296.1123386876454333, -195.6683190004872301 ) ) ;
#49375=CARTESIAN_POINT ( 'NONE',  ( -6.535770833326606244, -290.4747575874213794, -201.5764878373796307 ) ) ;
#49376=CARTESIAN_POINT ( 'NONE',  ( -92.81208482793789472, -291.2839303038761045, -216.8808019135353504 ) ) ;
#49377=CARTESIAN_POINT ( 'NONE',  ( -2.299288039690894792, -278.5896319226638411, -336.8596727356722340 ) ) ;
#49378=CARTESIAN_POINT ( 'NONE',  ( -38.07709782766258400, -272.0427788392063349, -195.3647191135007972 ) ) ;
#49380=CARTESIAN_POINT ( 'NONE',  ( 1.377635955367124465, -284.4592333065026537, -335.2466110531629511 ) ) ;
#49382=CARTESIAN_POINT ( 'NONE',  ( -110.1424918677905396, -282.7841634197175154, -252.2796705929992811 ) ) ;
#49383=SHAPE_REPRESENTATION ( 'High-Pressure Air Hose', ( #18940 ), #6864 ) ;
#49385=CARTESIAN_POINT ( 'NONE',  ( -67.47217027397731215, -294.2513306055011526, -337.3023629795414422 ) ) ;
#49386=CARTESIAN_POINT ( 'NONE',  ( 33.48507799939267926, -285.9835405036366183, -292.7678768272236880 ) ) ;
#49388=CARTESIAN_POINT ( 'NONE',  ( 4.923005535238533348, -292.4808522086966605, -332.3183233885110894 ) ) ;
#49389=CARTESIAN_POINT ( 'NONE',  ( -107.5964409500042649, -282.6479794078484815, -300.2785676423941368 ) ) ;
#49390=CARTESIAN_POINT ( 'NONE',  ( -16.71745902260857264, -281.9231969900390027, -199.5015308242051333 ) ) ;
#49391=CARTESIAN_POINT ( 'NONE',  ( -113.9302915993236667, -285.7976385458368327, -267.1464569531382836 ) ) ;
#49392=CARTESIAN_POINT ( 'NONE',  ( 36.20529224966779225, -280.0342637357871354, -289.4612208169772316 ) ) ;
#49393=CARTESIAN_POINT ( 'NONE',  ( 31.84059427389619756, -287.2426492264644935, -247.0628317520643407 ) ) ;
#49395=CARTESIAN_POINT ( 'NONE',  ( -104.8043604735452163, -279.5838067122942334, -299.8854042964910604 ) ) ;
#49396=CARTESIAN_POINT ( 'NONE',  ( -92.84247536346586571, -278.6777971285011972, -318.0294059278054419 ) ) ;
#49397=CARTESIAN_POINT ( 'NONE',  ( -4.235222826569365218, -288.4662586103927993, -202.6537132561683734 ) ) ;
#49399=CARTESIAN_POINT ( 'NONE',  ( -99.92031302022661521, -296.9800116850897780, -225.4955720367904917 ) ) ;
#49400=CARTESIAN_POINT ( 'NONE',  ( 15.25994442785172289, -290.2846324905020765, -323.3225548165859777 ) ) ;
#49403=CARTESIAN_POINT ( 'NONE',  ( 44.71564893372296723, -278.0519495502701375, -270.3284710469131937 ) ) ;
#49405=CARTESIAN_POINT ( 'NONE',  ( 26.94804623675772248, -273.0300826965657848, -231.3147130844005233 ) ) ;
#49406=CARTESIAN_POINT ( 'NONE',  ( 14.91509961193351153, -292.7298278018279802, -325.8198169838761373 ) ) ;
#49407=CARTESIAN_POINT ( 'NONE',  ( -107.2916408948669869, -272.1835785270253041, -248.9534160687415749 ) ) ;
#49408=CARTESIAN_POINT ( 'NONE',  ( 33.75592638118311584, -289.3282176880996417, -289.9371406849874120 ) ) ;
#49409=CARTESIAN_POINT ( 'NONE',  ( 0.9046582555454086849, -282.3296963963192070, -206.9362727628315497 ) ) ;
#49410=CARTESIAN_POINT ( 'NONE',  ( -82.48977217368603476, -291.0807374593202326, -332.0073496755800306 ) ) ;
#49411=CARTESIAN_POINT ( 'NONE',  ( -93.22107755772663040, -291.1493789675248536, -322.6944440754704146 ) ) ;
#49412=CARTESIAN_POINT ( 'NONE',  ( -96.68368674968338894, -285.9235182862970532, -316.2463218228793949 ) ) ;
#49413=CARTESIAN_POINT ( 'NONE',  ( -28.22710978558685113, -280.3313216066584914, -193.8488492315136682 ) ) ;
#49414=CARTESIAN_POINT ( 'NONE',  ( -16.92002158697798109, -292.8704321592006750, -343.1632966093561663 ) ) ;
#49415=CARTESIAN_POINT ( 'NONE',  ( 36.98556796121964396, -281.1330518979061708, -250.1999894972327070 ) ) ;
#49416=CARTESIAN_POINT ( 'NONE',  ( 36.05947611051713153, -277.2675187611154684, -259.1792451408117586 ) ) ;
#49417=CARTESIAN_POINT ( 'NONE',  ( 17.40634833298267736, -284.6948066931273047, -313.9805196606274080 ) ) ;
#49418=CARTESIAN_POINT ( 'NONE',  ( 20.04010931073992552, -274.4743582386694243, -320.1934725044154675 ) ) ;
#49420=CARTESIAN_POINT ( 'NONE',  ( 15.30807541936421678, -280.3283352732976255, -219.6332399031979890 ) ) ;
#49421=CARTESIAN_POINT ( 'NONE',  ( -39.93406478367798940, -278.2890813930548575, -346.9331684537138472 ) ) ;
#49422=CARTESIAN_POINT ( 'NONE',  ( -35.39393116032591280, -275.3922497951883201, -196.8811905241217062 ) ) ;
#49423=CARTESIAN_POINT ( 'NONE',  ( -29.47509650015330251, -285.2082409720796363, -194.0005472665238244 ) ) ;
#49424=CARTESIAN_POINT ( 'NONE',  ( -111.3820781893685137, -292.3370658619879805, -268.4577588059781874 ) ) ;
#49425=CARTESIAN_POINT ( 'NONE',  ( -97.19745026043671032, -274.7895696984243727, -223.2046805135603904 ) ) ;
#49427=CARTESIAN_POINT ( 'NONE',  ( -66.05776078182081790, -274.9993079865130881, -199.4338074242330947 ) ) ;
#49430=CARTESIAN_POINT ( 'NONE',  ( -112.0438826179248366, -298.6093062999666472, -265.9325340999852187 ) ) ;
#49431=CARTESIAN_POINT ( 'NONE',  ( -110.7835259300970279, -282.3671488988025544, -284.7251930423820454 ) ) ;
#49432=CARTESIAN_POINT ( 'NONE',  ( -99.18507155737479764, -290.8286594947131789, -224.5008257068041644 ) ) ;
#49433=CARTESIAN_POINT ( 'NONE',  ( 26.69966959923290872, -273.0552622143658255, -231.9131996019850703 ) ) ;
#49434=CARTESIAN_POINT ( 'NONE',  ( -4.657533988044860962, -290.2289052117240544, -339.2099297022812152 ) ) ;
#49435=CARTESIAN_POINT ( 'NONE',  ( -52.41997561662444127, -290.7749421919414772, -198.5672983850029993 ) ) ;
#49437=CARTESIAN_POINT ( 'NONE',  ( -112.5565452629291912, -288.9562423503023183, -283.9011273403303335 ) ) ;
#49438=CARTESIAN_POINT ( 'NONE',  ( -107.7711572187402140, -290.4735449506566738, -251.0795448945729049 ) ) ;
#49440=CARTESIAN_POINT ( 'NONE',  ( 0.1207374816257044542, -287.6184339904154399, -203.4278364882096639 ) ) ;
#49441=CARTESIAN_POINT ( 'NONE',  ( -105.2859206908969298, -278.5277770804569855, -297.1131343331007315 ) ) ;
#49442=CARTESIAN_POINT ( 'NONE',  ( -4.646843621756564069, -293.5518285725733563, -339.7479930571689124 ) ) ;
#49443=CARTESIAN_POINT ( 'NONE',  ( -63.86905923309991806, -284.0405893864820541, -342.5387599876568174 ) ) ;
#49444=CARTESIAN_POINT ( 'NONE',  ( -109.0103503931437814, -285.2432960619930782, -242.1207800228139035 ) ) ;
#49445=CARTESIAN_POINT ( 'NONE',  ( 30.35571859035506037, -282.2518552521718789, -297.7316675854043524 ) ) ;
#49446=CARTESIAN_POINT ( 'NONE',  ( -56.14975209998562633, -169.4529236618342622, -364.5118392738439752 ) ) ;
#49447=CARTESIAN_POINT ( 'NONE',  ( 63.42894017176210752, 48.18213374631179136, -317.6803299212049865 ) ) ;
#49448=CARTESIAN_POINT ( 'NONE',  ( -103.1447046786039579, -253.6660498445109226, -324.1576556378894907 ) ) ;
#49449=CARTESIAN_POINT ( 'NONE',  ( -38.07374021736068670, -273.2399129551845363, -197.2033033293363644 ) ) ;
#49450=CARTESIAN_POINT ( 'NONE',  ( -13.95386475250040093, -273.2831936092418914, -200.8828103631724105 ) ) ;
#49451=CARTESIAN_POINT ( 'NONE',  ( -98.22960625220127895, -295.4315019411887420, -317.3950396915814736 ) ) ;
#49452=CARTESIAN_POINT ( 'NONE',  ( -69.19725544157302011, -196.5455075490810657, -357.0703453118406969 ) ) ;
#49453=CARTESIAN_POINT ( 'NONE',  ( -103.7928402092161235, -271.7338217202679971, -232.3398782779615601 ) ) ;
#49454=CARTESIAN_POINT ( 'NONE',  ( -97.10864016964349332, -299.0196190437834503, -226.3080874927117918 ) ) ;
#49455=CARTESIAN_POINT ( 'NONE',  ( -106.0049828406917101, -291.9747131526716544, -244.5347177229220392 ) ) ;
#49457=CARTESIAN_POINT ( 'NONE',  ( -73.18147670076969291, -298.5304458648267314, -202.4177599501777536 ) ) ;
#49458=CARTESIAN_POINT ( 'NONE',  ( 33.08691790676105171, -287.7878789450689965, -250.9240862264044836 ) ) ;
#49459=CARTESIAN_POINT ( 'NONE',  ( -11.10271919309420063, -295.5216593545654860, -342.6371999761510665 ) ) ;
#49460=CARTESIAN_POINT ( 'NONE',  ( -3.250406724806273129, -295.1064021985593513, -339.3489709049057410 ) ) ;
#49461=CARTESIAN_POINT ( 'NONE',  ( 33.11725889488988628, -293.9716102246571268, -289.5014533879905230 ) ) ;
#49462=ORIENTED_EDGE ( 'NONE', *, *, #2914, .F. ) ;
#49463=CARTESIAN_POINT ( 'NONE',  ( 36.80095384282484616, -277.2866570656211707, -255.7946818047045952 ) ) ;
#49465=CARTESIAN_POINT ( 'NONE',  ( -71.20185806225903491, -279.1247490881081035, -201.2740959868586117 ) ) ;
#49466=CARTESIAN_POINT ( 'NONE',  ( -16.58541738105294172, -275.2681287427270718, -200.0758771524112660 ) ) ;
#49467=CARTESIAN_POINT ( 'NONE',  ( 6.630096824065898176, -276.4006525444441991, -208.3251524675641519 ) ) ;
#49468=CARTESIAN_POINT ( 'NONE',  ( 24.69806964495408153, -274.1503487569419804, -313.2237394437113949 ) ) ;
#49469=CARTESIAN_POINT ( 'NONE',  ( -68.09796366834507353, -298.2887424294363541, -204.0304306133187993 ) ) ;
#49470=CARTESIAN_POINT ( 'NONE',  ( -103.3043138675389514, -294.6868285965343830, -303.1000690853238666 ) ) ;
#49472=CARTESIAN_POINT ( 'NONE',  ( -112.0276974366332894, -279.2764862227519416, -251.8265517239939300 ) ) ;
#49473=CARTESIAN_POINT ( 'NONE',  ( 33.24273632964369796, -275.9647500860138507, -288.9846873093779891 ) ) ;
#49474=CARTESIAN_POINT ( 'NONE',  ( 37.80894475152727807, -286.0564668012131051, -256.0196101091842706 ) ) ;
#49475=CARTESIAN_POINT ( 'NONE',  ( 28.74821194883168118, -300.8778160839800648, -195.1719723918581053 ) ) ;
#49477=CARTESIAN_POINT ( 'NONE',  ( 26.51329963375439291, -286.2607146584775819, -234.5483269106472903 ) ) ;
#49478=CARTESIAN_POINT ( 'NONE',  ( -2.654609909276719915, -278.7572074108526863, -204.9649413578463566 ) ) ;
#49479=CARTESIAN_POINT ( 'NONE',  ( -27.46143780333180828, -278.7547148109621844, -197.3865714288429274 ) ) ;
#49480=CARTESIAN_POINT ( 'NONE',  ( -92.75298635848811557, -281.9342016311511543, -320.0884899109427693 ) ) ;
#49481=CARTESIAN_POINT ( 'NONE',  ( 36.83476319661841814, -289.4056295124209441, -258.9370324115632798 ) ) ;
#49482=CARTESIAN_POINT ( 'NONE',  ( -74.19947292626356727, -278.7589510638653678, -333.8326477372087879 ) ) ;
#49484=CARTESIAN_POINT ( 'NONE',  ( -101.2569455388316726, -276.2445639505675672, -311.5523723529313429 ) ) ;
#49485=CARTESIAN_POINT ( 'NONE',  ( 22.35929229859623746, -275.6152737403278934, -228.1531491960829214 ) ) ;
#49486=CARTESIAN_POINT ( 'NONE',  ( 37.35778549759002942, -283.4392933612969045, -261.5392256303246654 ) ) ;
#49488=CARTESIAN_POINT ( 'NONE',  ( -10.06001275522469740, -290.6188696538366116, -340.8240425048663269 ) ) ;
#49489=CARTESIAN_POINT ( 'NONE',  ( -28.96227084160118892, -290.1580768956535508, -195.7791394156632521 ) ) ;
#49491=CARTESIAN_POINT ( 'NONE',  ( 82.15009695330279271, -299.4571376875543365, -197.3638982236675190 ) ) ;
#49492=CARTESIAN_POINT ( 'NONE',  ( -62.18072331723876545, -272.4070535918263545, -201.1927263230633116 ) ) ;
#49493=CARTESIAN_POINT ( 'NONE',  ( 36.94389710783553937, -291.6972964711824261, -270.7903160613001319 ) ) ;
#49494=CARTESIAN_POINT ( 'NONE',  ( -105.6472514815422983, -266.3687386123619376, -319.2208520127341558 ) ) ;
#49496=CARTESIAN_POINT ( 'NONE',  ( -112.4542890685213763, -288.8614080061461777, -283.8814648792027242 ) ) ;
#49497=CARTESIAN_POINT ( 'NONE',  ( -76.53490712612479285, -285.1857482956578451, -332.9542000552448826 ) ) ;
#49498=CARTESIAN_POINT ( 'NONE',  ( -65.52470493161366960, -284.8532835358356579, -338.3534474379856078 ) ) ;
#49499=CARTESIAN_POINT ( 'NONE',  ( -76.20425608541822271, -284.3885809887270852, -332.4073438537532184 ) ) ;
#49500=CARTESIAN_POINT ( 'NONE',  ( -89.66245974754967563, -293.2991109728522474, -216.0581949996354751 ) ) ;
#49501=CARTESIAN_POINT ( 'NONE',  ( 37.88615260635930326, -273.5349981528704575, -262.7501664701212007 ) ) ;
#49502=CARTESIAN_POINT ( 'NONE',  ( 37.92382025403457391, -275.6826096186777590, -254.1480993044922911 ) ) ;
#49503=CARTESIAN_POINT ( 'NONE',  ( -111.9423063141627352, -288.4790296920276091, -282.3637741688511369 ) ) ;
#49504=CARTESIAN_POINT ( 'NONE',  ( -39.96295261462560688, -277.0842004637141258, -347.3295545798556532 ) ) ;
#49505=CARTESIAN_POINT ( 'NONE',  ( -50.74228749793972071, -297.2040775523693128, -343.7932026459827739 ) ) ;
#49508=CARTESIAN_POINT ( 'NONE',  ( -109.2057938497800933, -283.0345584545727888, -285.8091130482690119 ) ) ;
#49509=CARTESIAN_POINT ( 'NONE',  ( -91.60857109470765636, -277.2794066226040854, -218.5171905846226821 ) ) ;
#49511=CARTESIAN_POINT ( 'NONE',  ( 11.35821897250883339, -273.1926209672289474, -211.5470117345105336 ) ) ;
#49512=CARTESIAN_POINT ( 'NONE',  ( -13.76035386816042028, -276.0865810103486524, -339.6083501210218856 ) ) ;
#49513=CARTESIAN_POINT ( 'NONE',  ( 1.955781103605104709, -296.0363515956383367, -332.7626873915692158 ) ) ;
#49514=CARTESIAN_POINT ( 'NONE',  ( 39.40119774083780868, -280.4672661272284131, -269.9457209600016654 ) ) ;
#49515=CARTESIAN_POINT ( 'NONE',  ( -26.15969492799074558, -295.8475481464012660, -342.7377109343363486 ) ) ;
#49516=CARTESIAN_POINT ( 'NONE',  ( -108.9698912448646269, -297.5233737609799505, -297.3935862412163829 ) ) ;
#49517=CARTESIAN_POINT ( 'NONE',  ( -35.81345161516997422, -297.9051277492375789, -197.3611626661092657 ) ) ;
#49518=CARTESIAN_POINT ( 'NONE',  ( -78.36997468091350072, -293.5002010129019254, -207.5783071637992521 ) ) ;
#49519=CARTESIAN_POINT ( 'NONE',  ( -46.50760314449774313, -286.1055498940846178, -193.9086083678337218 ) ) ;
#49520=CARTESIAN_POINT ( 'NONE',  ( -32.73366931883641229, -272.2492001938284147, -194.7236352448972525 ) ) ;
#49521=CARTESIAN_POINT ( 'NONE',  ( 2.742822895989173393, -286.4076286265218414, -204.6174413403601022 ) ) ;
#49522=CARTESIAN_POINT ( 'NONE',  ( -100.8807796076376775, -281.0614440071479407, -231.0880770847348913 ) ) ;
#49523=CARTESIAN_POINT ( 'NONE',  ( -91.68780161778320803, -284.3124121309485304, -221.1957865600609523 ) ) ;
#49524=CARTESIAN_POINT ( 'NONE',  ( -34.76180697620001325, -287.0195713852256745, -345.3167368700294446 ) ) ;
#49525=CARTESIAN_POINT ( 'NONE',  ( -69.18520112214993389, -196.4157418647702968, -356.4528236438462159 ) ) ;
#49526=CARTESIAN_POINT ( 'NONE',  ( -2.151243864010800699, -286.0386496698555447, -206.2760749116829118 ) ) ;
#49527=CARTESIAN_POINT ( 'NONE',  ( -113.8789064103646780, -289.5286037834381432, -276.9215164603783137 ) ) ;
#49528=CARTESIAN_POINT ( 'NONE',  ( -106.8380299810364562, -279.7474731427586789, -301.7416430411084320 ) ) ;
#49530=CARTESIAN_POINT ( 'NONE',  ( -109.2673725027800202, -279.5340802466330388, -296.5927324422127640 ) ) ;
#49531=CARTESIAN_POINT ( 'NONE',  ( 21.81069152926886900, -281.9841633384567103, -313.1609556136323249 ) ) ;
#49532=CARTESIAN_POINT ( 'NONE',  ( 36.59306450925804910, -277.3896077751226130, -257.6893042480007239 ) ) ;
#49533=CARTESIAN_POINT ( 'NONE',  ( 11.19831191540491311, -294.4013019165051332, -330.2032949994159594 ) ) ;
#49534=CARTESIAN_POINT ( 'NONE',  ( -64.44102773373909088, -287.4275611035830593, -339.9684785925542769 ) ) ;
#49535=CARTESIAN_POINT ( 'NONE',  ( -98.69878289298003438, -296.0272434787479483, -230.1502765364316474 ) ) ;
#49538=CARTESIAN_POINT ( 'NONE',  ( -64.55956109852400004, -285.3304219374083459, -339.6467748141643597 ) ) ;
#49539=CARTESIAN_POINT ( 'NONE',  ( -50.47917533872814744, -294.8912765312112469, -342.1907374426260162 ) ) ;
#49540=CARTESIAN_POINT ( 'NONE',  ( 37.77063626484817149, -294.8261971509081718, -285.8410867322615445 ) ) ;
#49541=CARTESIAN_POINT ( 'NONE',  ( -67.81931484460747583, -284.1145029419897696, -336.8066420584136154 ) ) ;
#49542=CARTESIAN_POINT ( 'NONE',  ( -38.34228576782813036, -273.0986494635421877, -193.6029324753430103 ) ) ;
#49543=CARTESIAN_POINT ( 'NONE',  ( 5.507411626225722223, -289.1397416561646878, -334.2145940682265746 ) ) ;
#49544=CARTESIAN_POINT ( 'NONE',  ( -47.12077928171004260, -281.3147074676109582, -345.4921707492155178 ) ) ;
#49545=CARTESIAN_POINT ( 'NONE',  ( -109.4555248953025028, -291.2278475023503006, -243.2770414514255037 ) ) ;
#49546=CARTESIAN_POINT ( 'NONE',  ( 27.05111373861568680, -288.3559616659129574, -304.9020584416039696 ) ) ;
#49549=CARTESIAN_POINT ( 'NONE',  ( 153.3117529583858527, 204.6325910983726999, -214.2920792270980996 ) ) ;
#49550=CARTESIAN_POINT ( 'NONE',  ( -106.6379572354042296, -282.4809262143061233, -236.9535640164627353 ) ) ;
#49552=CARTESIAN_POINT ( 'NONE',  ( -57.18372481543556773, -278.7103655612335729, -199.7883177753582800 ) ) ;
#49553=CARTESIAN_POINT ( 'NONE',  ( 38.19881901303173777, -275.0335861821708363, -255.5498297369316276 ) ) ;
#49554=CARTESIAN_POINT ( 'NONE',  ( -43.32900050412526127, -279.1281170140257473, -344.9545537593516542 ) ) ;
#49555=CARTESIAN_POINT ( 'NONE',  ( -96.95435030675994881, -248.2403463976193621, -332.6261155525420463 ) ) ;
#49556=CARTESIAN_POINT ( 'NONE',  ( 21.52843624158481362, -279.4670369831338235, -221.6485596558759994 ) ) ;
#49557=CARTESIAN_POINT ( 'NONE',  ( -69.74548977179161113, -281.5010251890507789, -337.6198718618985595 ) ) ;
#49558=CARTESIAN_POINT ( 'NONE',  ( -91.95294407782000690, -297.5787675882438634, -323.1965800079927931 ) ) ;
#49559=CARTESIAN_POINT ( 'NONE',  ( 8.271472623199930041, -294.9011670952120312, -327.5000151657403080 ) ) ;
#49560=ORIENTED_EDGE ( 'NONE', *, *, #39491, .T. ) ;
#49561=CARTESIAN_POINT ( 'NONE',  ( -110.2809895493547998, -289.1189689047381535, -279.3668681743888556 ) ) ;
#49562=CARTESIAN_POINT ( 'NONE',  ( -2.611013291941904235, -275.1506583338693304, -201.7381837791727435 ) ) ;
#49563=CARTESIAN_POINT ( 'NONE',  ( -41.87046271344525650, -298.1601761463480216, -197.5017307084477238 ) ) ;
#49564=ORIENTED_EDGE ( 'NONE', *, *, #43456, .T. ) ;
#49568=CARTESIAN_POINT ( 'NONE',  ( -64.94520369595728937, -280.7625471628977607, -202.4474031323467500 ) ) ;
#49569=CARTESIAN_POINT ( 'NONE',  ( 3.261310291122220928, -282.3494526346327689, -206.0699364363243262 ) ) ;
#49570=CARTESIAN_POINT ( 'NONE',  ( -73.92469122968472561, -282.6092327882400355, -333.8625342478071047 ) ) ;
#49571=CARTESIAN_POINT ( 'NONE',  ( 19.77148438193743729, -282.7509526114511118, -222.9183055582599877 ) ) ;
#49572=CARTESIAN_POINT ( 'NONE',  ( 31.90669141675908804, -274.3664828682270809, -295.7158029609094569 ) ) ;
#49575=CARTESIAN_POINT ( 'NONE',  ( -14.62765082341001310, -277.5680316141420576, -343.8213981323971780 ) ) ;
#49579=CARTESIAN_POINT ( 'NONE',  ( -35.90472487002985957, -285.0141347437764239, -345.7154563273417693 ) ) ;
#49580=CARTESIAN_POINT ( 'NONE',  ( -1.167960896321708075, -291.7424252701682690, -206.7536673425425420 ) ) ;
#49581=CARTESIAN_POINT ( 'NONE',  ( 0.6616879887054784026, -287.9082371396405620, -337.2722809867586875 ) ) ;
#49582=CARTESIAN_POINT ( 'NONE',  ( -84.27335583830985399, -283.6365492073206269, -213.0634882587885102 ) ) ;
#49583=CARTESIAN_POINT ( 'NONE',  ( -60.14411520869510497, -284.3254146904577624, -200.3938057380328814 ) ) ;
#49584=CARTESIAN_POINT ( 'NONE',  ( -98.19466404581379493, -288.2128417990739422, -312.5128459672343411 ) ) ;
#49585=CARTESIAN_POINT ( 'NONE',  ( -42.94801503898276707, -284.3294240698869544, -343.5941236076088217 ) ) ;
#49586=CARTESIAN_POINT ( 'NONE',  ( 34.67285453171767529, -273.2801550712969743, -249.2293634457164728 ) ) ;
#49587=CARTESIAN_POINT ( 'NONE',  ( -113.5554106382944468, -282.9211639783850387, -272.8030521181833592 ) ) ;
#49588=CARTESIAN_POINT ( 'NONE',  ( -82.94830302127458310, -297.6758264042525752, -329.9668054032773057 ) ) ;
#49589=CARTESIAN_POINT ( 'NONE',  ( -13.26622357517111617, -284.3639863414972524, -199.1543777550592722 ) ) ;
#49590=CARTESIAN_POINT ( 'NONE',  ( -108.2032837142395749, -279.7373841354975639, -251.8173843365363211 ) ) ;
#49591=CARTESIAN_POINT ( 'NONE',  ( 17.00785990269967840, -288.8241946479862463, -218.3615801760174122 ) ) ;
#49594=CARTESIAN_POINT ( 'NONE',  ( 25.33126874728590039, -296.0389554458250245, -312.5679085555575512 ) ) ;
#49595=CARTESIAN_POINT ( 'NONE',  ( -109.9012063239138683, -276.7964472443777026, -251.3339455880679338 ) ) ;
#49596=CARTESIAN_POINT ( 'NONE',  ( -95.53192449113932128, -290.4285580735957524, -220.1607689647812833 ) ) ;
#49597=CARTESIAN_POINT ( 'NONE',  ( 25.09330174392906798, -292.4908341288756901, -309.8056540410530033 ) ) ;
#49598=CARTESIAN_POINT ( 'NONE',  ( -35.63466596294345123, -278.7588033778637282, -196.8753064768455658 ) ) ;
#49599=CARTESIAN_POINT ( 'NONE',  ( -78.17190898149146960, -295.6367116617522584, -208.3012988245606891 ) ) ;
#49600=CARTESIAN_POINT ( 'NONE',  ( -79.82936358749519457, -292.7796340671091571, -210.3317237195485916 ) ) ;
#49601=CARTESIAN_POINT ( 'NONE',  ( -69.91165696735023971, -282.1233781216988064, -202.8022627189028810 ) ) ;
#49602=CARTESIAN_POINT ( 'NONE',  ( -104.0066924283642322, -294.5451093671936746, -307.5971586733796812 ) ) ;
#49603=CARTESIAN_POINT ( 'NONE',  ( -58.90361246526235561, -290.9357826069282282, -340.9944099585647450 ) ) ;
#49604=CARTESIAN_POINT ( 'NONE',  ( 19.63394104791870731, -291.1019812454345583, -220.0647154533644994 ) ) ;
#49605=CARTESIAN_POINT ( 'NONE',  ( -75.29896657940909677, -292.9610962875026985, -207.2570240953997143 ) ) ;
#49607=CARTESIAN_POINT ( 'NONE',  ( -110.4671951191295989, -291.3080536491619910, -273.9269992693220388 ) ) ;
#49610=CARTESIAN_POINT ( 'NONE',  ( -99.71669408052348160, -292.3492262705923963, -225.8935022547664460 ) ) ;
#49611=CARTESIAN_POINT ( 'NONE',  ( 34.89456460024948115, -279.8493962182371888, -291.9956943013424961 ) ) ;
#49612=CARTESIAN_POINT ( 'NONE',  ( 34.06757603069395657, -293.7528807033340854, -285.5774379089120885 ) ) ;
#49613=CARTESIAN_POINT ( 'NONE',  ( 33.17294455255802887, -281.1576968875261855, -239.4307949069247172 ) ) ;
#49614=CARTESIAN_POINT ( 'NONE',  ( 39.50776930507541351, -281.2852057226770057, -275.6636721458789907 ) ) ;
#49615=CARTESIAN_POINT ( 'NONE',  ( 8.159987322417903144, -284.6737996474529950, -210.6750414418727928 ) ) ;
#49616=CARTESIAN_POINT ( 'NONE',  ( 35.14141974038829375, -279.8997213074912338, -286.3942966432434787 ) ) ;
#49617=CARTESIAN_POINT ( 'NONE',  ( -59.88388321257586000, -283.7600525532362212, -198.7748273930347693 ) ) ;
#49619=CARTESIAN_POINT ( 'NONE',  ( -35.33468722438668408, -278.5567669666513666, -194.0678292584169640 ) ) ;
#49620=CARTESIAN_POINT ( 'NONE',  ( -64.42511264268087245, -284.6271620021917101, -198.5975743485952023 ) ) ;
#49621=CARTESIAN_POINT ( 'NONE',  ( -31.33662544711657461, -274.9327347012768428, -197.4338273301233073 ) ) ;
#49623=CARTESIAN_POINT ( 'NONE',  ( 17.31711840160693328, -294.4487299873505322, -220.6993588358198508 ) ) ;
#49624=CARTESIAN_POINT ( 'NONE',  ( 39.04135970047725124, -276.9514893513464813, -268.3033370053312865 ) ) ;
#49625=CARTESIAN_POINT ( 'NONE',  ( -100.6032727243791811, -277.7177423027198984, -306.9326810004016011 ) ) ;
#49626=CARTESIAN_POINT ( 'NONE',  ( -113.1329248472795399, -290.5479374808705302, -284.0256608303066059 ) ) ;
#49627=CARTESIAN_POINT ( 'NONE',  ( -1.790921918066832985, -278.5992873217503529, -203.6868623150331246 ) ) ;
#49628=CARTESIAN_POINT ( 'NONE',  ( -27.84698658338809096, -292.0027258700518473, -193.8950725848873162 ) ) ;
#49629=EDGE_CURVE ( 'NONE', #31036, #14296, #64991, .T. ) ;
#49630=CARTESIAN_POINT ( 'NONE',  ( -98.48941110709382940, -290.1691730303283521, -229.9656015824488406 ) ) ;
#49631=CARTESIAN_POINT ( 'NONE',  ( -1.680188893756997093, -292.5794578047132291, -336.3548329139419479 ) ) ;
#49634=CARTESIAN_POINT ( 'NONE',  ( 6.718338184219007303, -292.1777447237187175, -212.0798905985906515 ) ) ;
#49636=CARTESIAN_POINT ( 'NONE',  ( -105.5937364680635966, -275.8380690714489560, -285.9065529553535612 ) ) ;
#49637=CARTESIAN_POINT ( 'NONE',  ( -100.5500932208516929, -296.1880342579137846, -226.7774985727764658 ) ) ;
#49638=CARTESIAN_POINT ( 'NONE',  ( -83.57180211223099775, -284.9862033013532709, -331.3872817576119019 ) ) ;
#49639=CARTESIAN_POINT ( 'NONE',  ( 34.99643936965391333, -287.2512179996217014, -260.1839862995061594 ) ) ;
#49640=CARTESIAN_POINT ( 'NONE',  ( 33.52141173430761967, -276.8052013668915379, -249.9520608366478598 ) ) ;
#49641=CARTESIAN_POINT ( 'NONE',  ( -95.23384881368116339, -293.9198106378700572, -317.5017610726400221 ) ) ;
#49642=CARTESIAN_POINT ( 'NONE',  ( -107.6766929757261266, -298.6158341756103027, -247.1558544014971233 ) ) ;
#49643=CARTESIAN_POINT ( 'NONE',  ( -7.359414719053728682, -275.4448656147606016, -337.3550958277109544 ) ) ;
#49646=CARTESIAN_POINT ( 'NONE',  ( -114.2883800339493945, -296.2642707458900873, -266.7320425566662152 ) ) ;
#49647=CARTESIAN_POINT ( 'NONE',  ( 32.31355466127269693, -289.1269743330070128, -243.9581742184847997 ) ) ;
#49648=CARTESIAN_POINT ( 'NONE',  ( -71.68231431399064491, -295.5982969377303107, -203.6706444086711656 ) ) ;
#49650=CARTESIAN_POINT ( 'NONE',  ( 24.32878666437833104, -288.7455111955325719, -309.6121527064545376 ) ) ;
#49652=CARTESIAN_POINT ( 'NONE',  ( -94.77775522932822128, -278.3030756798927996, -219.4305791311844871 ) ) ;
#49653=CARTESIAN_POINT ( 'NONE',  ( 21.29530990945289659, -294.8750403548178838, -320.1106289427427782 ) ) ;
#49654=CARTESIAN_POINT ( 'NONE',  ( -97.19856780072755953, -288.0613605313578773, -316.8095934867362757 ) ) ;
#49655=CARTESIAN_POINT ( 'NONE',  ( -66.91239187261079735, -295.7624826590495672, -341.4479435667584539 ) ) ;
#49656=CARTESIAN_POINT ( 'NONE',  ( 35.72916729967085558, -293.8906406244881282, -270.7558028428315424 ) ) ;
#49660=CARTESIAN_POINT ( 'NONE',  ( -48.74608349352957504, -290.7148443258338943, -345.8642122658699236 ) ) ;
#49661=CARTESIAN_POINT ( 'NONE',  ( -115.3288506153726871, -280.8376638359844151, -288.1938231032136741 ) ) ;
#49662=CARTESIAN_POINT ( 'NONE',  ( -84.49787322702056258, -278.7709811839317240, -209.5515938806253189 ) ) ;
#49663=CARTESIAN_POINT ( 'NONE',  ( -104.6508006407196802, -286.1190163151418915, -303.1834571744745972 ) ) ;
#49664=CARTESIAN_POINT ( 'NONE',  ( 22.54152070417518772, -285.4866857326896366, -222.8786281705411625 ) ) ;
#49665=CARTESIAN_POINT ( 'NONE',  ( 35.93496382104577691, -285.8015801664035394, -283.4700737045235428 ) ) ;
#49666=CARTESIAN_POINT ( 'NONE',  ( 18.97519612362179586, -278.1118691077887206, -321.0630098132747889 ) ) ;
#49667=CARTESIAN_POINT ( 'NONE',  ( -93.94052838712022435, -279.2047528621832839, -224.2571849648247735 ) ) ;
#49668=CARTESIAN_POINT ( 'NONE',  ( 29.06875212512782625, -280.4876672165820537, -239.6858164139459575 ) ) ;
#49669=CARTESIAN_POINT ( 'NONE',  ( 1.028806970584595248, -275.6313910885928635, -203.9441133298500688 ) ) ;
#49670=CARTESIAN_POINT ( 'NONE',  ( -101.5499708662807166, -277.8996932533872268, -228.4882948711697850 ) ) ;
#49671=CARTESIAN_POINT ( 'NONE',  ( -40.74239786503150640, -139.1097897353693043, -361.8818269458895998 ) ) ;
#49672=CARTESIAN_POINT ( 'NONE',  ( -29.87373460061922970, -275.0857525414263591, -193.9605309191074412 ) ) ;
#49673=CARTESIAN_POINT ( 'NONE',  ( -106.2257198045210771, -274.4969280293119596, -237.5327829029802444 ) ) ;
#49674=CARTESIAN_POINT ( 'NONE',  ( -114.2704648735229114, -287.0519495502703080, -270.3937649182068981 ) ) ;
#49677=CARTESIAN_POINT ( 'NONE',  ( 82.62056641594917039, -301.7796436375890039, -194.2090517697148186 ) ) ;
#49678=CARTESIAN_POINT ( 'NONE',  ( -2.049596653466665863, -287.6104143716297585, -206.0492558786767461 ) ) ;
#49679=CARTESIAN_POINT ( 'NONE',  ( -52.00005431648487075, -287.6273099305882965, -195.7480235018652195 ) ) ;
#49680=CARTESIAN_POINT ( 'NONE',  ( -18.45515703022170939, -288.1510543174051122, -341.0338234723051301 ) ) ;
#49681=CARTESIAN_POINT ( 'NONE',  ( -88.28548820939360553, -283.2506877295736558, -328.0886325323236292 ) ) ;
#49682=CARTESIAN_POINT ( 'NONE',  ( 25.83152688473413505, -279.4314095742582822, -232.1099269025458796 ) ) ;
#49683=CARTESIAN_POINT ( 'NONE',  ( -41.41398145405877074, -287.8607831278534945, -196.2249841810826751 ) ) ;
#49684=CARTESIAN_POINT ( 'NONE',  ( 33.40558350444596414, -279.7617100432004236, -249.7327488801840900 ) ) ;
#49685=CARTESIAN_POINT ( 'NONE',  ( -6.051555397364877464, -277.9472573267697157, -336.8743821977475363 ) ) ;
#49686=CARTESIAN_POINT ( 'NONE',  ( -11.47429486009469279, -274.8906215937448110, -201.9779292118369369 ) ) ;
#49687=CARTESIAN_POINT ( 'NONE',  ( 36.00076146474930994, -286.6265590629299709, -292.5175486488519709 ) ) ;
#49688=CARTESIAN_POINT ( 'NONE',  ( 23.28183560395387985, -282.9872311641152578, -317.5940955169109543 ) ) ;
#49689=CARTESIAN_POINT ( 'NONE',  ( -104.3603271607003080, -284.5525202608938571, -308.2583003458410076 ) ) ;
#49690=CARTESIAN_POINT ( 'NONE',  ( 35.35213792486316464, -281.6236964745351088, -263.1492342920464012 ) ) ;
#49694=CARTESIAN_POINT ( 'NONE',  ( -68.82211440461092877, -291.3219884770352337, -339.2903931898455880 ) ) ;
#49695=CARTESIAN_POINT ( 'NONE',  ( -100.9160869950618746, -272.1086698645432875, -233.9038964900763915 ) ) ;
#49696=CARTESIAN_POINT ( 'NONE',  ( 30.80817011324824861, -293.3609315278985719, -305.9828525328463797 ) ) ;
#49697=CARTESIAN_POINT ( 'NONE',  ( -110.1067658829752673, -288.8786206709077646, -282.1005037632070298 ) ) ;
#49698=CARTESIAN_POINT ( 'NONE',  ( 22.63890038393446602, -291.1934726271103386, -226.9771136712184330 ) ) ;
#49699=CARTESIAN_POINT ( 'NONE',  ( 28.59114552718344981, -289.1916847768924868, -302.6099996284083886 ) ) ;
#49700=CARTESIAN_POINT ( 'NONE',  ( -114.2704648735229114, -293.0519495502703080, -270.3937649182068981 ) ) ;
#49701=CARTESIAN_POINT ( 'NONE',  ( -103.3825209483136689, -292.0804366682577893, -305.9084193053351441 ) ) ;
#49702=CARTESIAN_POINT ( 'NONE',  ( -111.0747440640663655, -288.3639759312362116, -285.0369665777968748 ) ) ;
#49703=CARTESIAN_POINT ( 'NONE',  ( -83.50245649666280201, -293.4198109312240490, -211.1843974535695168 ) ) ;
#49704=CARTESIAN_POINT ( 'NONE',  ( -9.414723203474760993, -287.3675725798953522, -202.6460727989379507 ) ) ;
#49705=CARTESIAN_POINT ( 'NONE',  ( 34.93415448850418414, -295.2866542660498226, -249.6689545277754121 ) ) ;
#49706=CARTESIAN_POINT ( 'NONE',  ( -114.3276611901150659, -272.2616898454610350, -270.3574197013679168 ) ) ;
#49708=CARTESIAN_POINT ( 'NONE',  ( -111.9202768220849578, -274.6745027186147468, -259.2135409318198640 ) ) ;
#49710=CARTESIAN_POINT ( 'NONE',  ( -3.959231174534847408, -280.6116839024791716, -337.5222035863770884 ) ) ;
#49711=CARTESIAN_POINT ( 'NONE',  ( -113.4404092577192102, -295.8838235641732695, -259.6290520699915305 ) ) ;
#49712=CARTESIAN_POINT ( 'NONE',  ( 20.66346370439013214, -273.1518255304276863, -224.3693719893715581 ) ) ;
#49713=CARTESIAN_POINT ( 'NONE',  ( -51.57979615484179448, -275.3155206882368589, -343.4267789771403727 ) ) ;
#49714=CARTESIAN_POINT ( 'NONE',  ( -101.6541489594178671, -298.3501832310023474, -234.7921370840643362 ) ) ;
#49715=CARTESIAN_POINT ( 'NONE',  ( 17.67802907595304518, -273.3946276828778537, -217.2621713217016293 ) ) ;
#49716=CARTESIAN_POINT ( 'NONE',  ( -109.7183769884873783, -297.8024216431435320, -283.7346490028505741 ) ) ;
#49718=CARTESIAN_POINT ( 'NONE',  ( -101.6042868250468132, -296.8787084771199147, -305.3314150575736221 ) ) ;
#49720=CARTESIAN_POINT ( 'NONE',  ( 37.70702564139116220, -285.6590223072589083, -277.1504891859455597 ) ) ;
#49721=CARTESIAN_POINT ( 'NONE',  ( -65.57271514531647938, -297.6724027894083520, -203.0409145433498566 ) ) ;
#49722=CARTESIAN_POINT ( 'NONE',  ( -68.50075781982525314, -285.6539466809196597, -199.9328714335240136 ) ) ;
#49723=CARTESIAN_POINT ( 'NONE',  ( 37.12288259716916627, -287.4631987071650769, -289.8744521711566904 ) ) ;
#49724=CARTESIAN_POINT ( 'NONE',  ( -111.2798307700559377, -298.7187674465575924, -255.7495586203262690 ) ) ;
#49725=CARTESIAN_POINT ( 'NONE',  ( 24.43233675399941163, -292.1264055033022942, -312.6890782453603492 ) ) ;
#49726=CARTESIAN_POINT ( 'NONE',  ( -98.44172566682247805, -278.3720035304528437, -223.7462797582116139 ) ) ;
#49727=CARTESIAN_POINT ( 'NONE',  ( -95.99890600148557951, -287.4094976428776249, -317.0979686699210447 ) ) ;
#49729=CARTESIAN_POINT ( 'NONE',  ( 16.27496074099764201, -285.6297388381625524, -220.2188778058160779 ) ) ;
#49731=CARTESIAN_POINT ( 'NONE',  ( -81.60792948368583666, -287.6540168532412736, -330.9691453748866365 ) ) ;
#49732=CARTESIAN_POINT ( 'NONE',  ( -72.05916672277926693, -299.1851909532456943, -205.2227431646824982 ) ) ;
#49733=CARTESIAN_POINT ( 'NONE',  ( -11.72412971190821906, -281.8044268473148009, -198.3170543768111145 ) ) ;
#49734=CARTESIAN_POINT ( 'NONE',  ( -111.0027954374962889, -294.3692174197221902, -286.2497883133154346 ) ) ;
#49735=CARTESIAN_POINT ( 'NONE',  ( 3.390220919244847142, -282.4879635587228108, -331.0020504551936824 ) ) ;
#49736=CARTESIAN_POINT ( 'NONE',  ( -113.6020565022060964, -296.8531797794875047, -259.6187472219308461 ) ) ;
#49737=CARTESIAN_POINT ( 'NONE',  ( -110.9309288753746898, -273.9771951043131253, -270.3792229722685647 ) ) ;
#49738=CARTESIAN_POINT ( 'NONE',  ( -4.555522512807772983, -282.4842437307777345, -202.8927937204268517 ) ) ;
#49741=CARTESIAN_POINT ( 'NONE',  ( -97.06770705644282771, -296.2008161783655851, -227.9793702028909763 ) ) ;
#49743=DIRECTION ( 'NONE',  ( -1.000000000000000000, 0.000000000000000000, -0.000000000000000000 ) ) ;
#49744=CARTESIAN_POINT ( 'NONE',  ( -18.29207605295991712, -284.7855113607416797, -342.5878238165592506 ) ) ;
#49746=CARTESIAN_POINT ( 'NONE',  ( 31.98288692825983404, -284.6237833571634042, -237.0123917617631264 ) ) ;
#49747=CARTESIAN_POINT ( 'NONE',  ( 38.06226357854495035, -274.5641106988937850, -255.5827189383154803 ) ) ;
#49748=CARTESIAN_POINT ( 'NONE',  ( -4.831172163236261419, -292.3259308427347491, -204.9861529717488509 ) ) ;
#49749=CARTESIAN_POINT ( 'NONE',  ( 32.62886164679441237, -282.7662583247020507, -247.0740623273265442 ) ) ;
#49750=CARTESIAN_POINT ( 'NONE',  ( 16.19206890419980382, -277.8765737109999918, -321.1604879431225754 ) ) ;
#49751=CARTESIAN_POINT ( 'NONE',  ( -52.78067841596896415, -284.6713877280255360, -345.2499698865493087 ) ) ;
#49752=CARTESIAN_POINT ( 'NONE',  ( 32.35849621574372037, -280.0415000291916954, -247.2005414872594997 ) ) ;
#49753=CARTESIAN_POINT ( 'NONE',  ( -95.13123691389665737, -279.8924247039564079, -318.1867755589982494 ) ) ;
#49754=CARTESIAN_POINT ( 'NONE',  ( 76.38675318495047861, -299.4392170424915776, -193.3610342431294384 ) ) ;
#49755=CARTESIAN_POINT ( 'NONE',  ( 37.23821526959913086, -275.6251632670080767, -289.5140870422535500 ) ) ;
#49756=CARTESIAN_POINT ( 'NONE',  ( 21.30251398466877077, -294.8382676646551204, -224.4910585793413418 ) ) ;
#49757=CARTESIAN_POINT ( 'NONE',  ( 128.9467878515196162, -299.5541904835127980, -195.3611179825600175 ) ) ;
#49761=CARTESIAN_POINT ( 'NONE',  ( -113.0739147689394173, -294.7373817827403286, -266.7698167784902807 ) ) ;
#49762=CARTESIAN_POINT ( 'NONE',  ( -43.48104944718411247, -273.4803023304604039, -197.5072270856211105 ) ) ;
#49763=CARTESIAN_POINT ( 'NONE',  ( 38.96195801657260205, -295.0354543878029858, -267.4436248985124962 ) ) ;
#49764=CARTESIAN_POINT ( 'NONE',  ( 37.96971742631737357, -294.9342013471664359, -284.4391780805657959 ) ) ;
#49765=CARTESIAN_POINT ( 'NONE',  ( 35.80805840993487266, -289.7561556815304584, -286.2055236481873521 ) ) ;
#49766=CARTESIAN_POINT ( 'NONE',  ( -108.1719323841925871, -276.8668976351476658, -246.0545505532937796 ) ) ;
#49767=CARTESIAN_POINT ( 'NONE',  ( -29.53863327607716371, -278.8728663359054281, -344.4429308395170892 ) ) ;
#49768=CARTESIAN_POINT ( 'NONE',  ( -38.38655828616665389, -293.1451975357958872, -344.7937887181799965 ) ) ;
#49769=CARTESIAN_POINT ( 'NONE',  ( 38.05151388181356253, -283.5142879931343600, -278.3641237027651982 ) ) ;
#49770=CARTESIAN_POINT ( 'NONE',  ( -89.87480949249908235, -284.2094730787247272, -219.1561191593192461 ) ) ;
#49771=CARTESIAN_POINT ( 'NONE',  ( 204.9738562182569979, 293.9636489450776367, -54.00000000001201528 ) ) ;
#49773=CARTESIAN_POINT ( 'NONE',  ( -87.70601829063315336, -284.9914670230021443, -217.4884129000527651 ) ) ;
#49774=CARTESIAN_POINT ( 'NONE',  ( 24.01609537645098769, -283.2465998793716153, -316.3688721279685865 ) ) ;
#49775=CARTESIAN_POINT ( 'NONE',  ( -107.8676054081266500, -282.9629749341521006, -300.3984759287489510 ) ) ;
#49776=CARTESIAN_POINT ( 'NONE',  ( -96.64334107210639502, -280.1503675080806488, -221.5950525213766866 ) ) ;
#49777=CARTESIAN_POINT ( 'NONE',  ( -77.43399729802185050, -279.0993625569138317, -335.3479731977087681 ) ) ;
#49778=CARTESIAN_POINT ( 'NONE',  ( 7.450504543161046378, -296.9090924074130839, -326.4764044574609443 ) ) ;
#49779=CARTESIAN_POINT ( 'NONE',  ( -55.29403410364363225, -169.9286504849079904, -364.5147574933134251 ) ) ;
#49781=CARTESIAN_POINT ( 'NONE',  ( -106.0734115640449318, -274.9418047119115727, -240.6327310223400957 ) ) ;
#49782=CARTESIAN_POINT ( 'NONE',  ( -46.63682837063362996, -277.9538278851993027, -196.2450598393899668 ) ) ;
#49783=CARTESIAN_POINT ( 'NONE',  ( -74.20715666390071874, -293.3291786543345552, -203.9163128504025053 ) ) ;
#49784=CARTESIAN_POINT ( 'NONE',  ( 19.43019322377892166, -292.2498925517618318, -224.2886864290337030 ) ) ;
#49785=CARTESIAN_POINT ( 'NONE',  ( -68.03509219607683178, -288.9521356912331385, -340.9121107944810660 ) ) ;
#49787=CARTESIAN_POINT ( 'NONE',  ( -41.92847484860295282, -293.6834815892525512, -346.6860920940337110 ) ) ;
#49788=CARTESIAN_POINT ( 'NONE',  ( -73.93479024045835502, -283.9573723216579424, -206.2575723485693686 ) ) ;
#49789=CARTESIAN_POINT ( 'NONE',  ( -90.72068405743362973, -293.1456056904294769, -218.7709100491314302 ) ) ;
#49790=CARTESIAN_POINT ( 'NONE',  ( -23.95937649564948302, -284.1927967358367937, -342.6256105837574637 ) ) ;
#49792=CARTESIAN_POINT ( 'NONE',  ( -72.07655293769614957, -292.5454155814339856, -201.8899322832148471 ) ) ;
#49793=CARTESIAN_POINT ( 'NONE',  ( -7.980464836452424215, -280.9398203629957607, -203.4452201630073773 ) ) ;
#49794=CARTESIAN_POINT ( 'NONE',  ( 8.655424666131757760, -293.2322592690497913, -331.6169195703292871 ) ) ;
#49795=CARTESIAN_POINT ( 'NONE',  ( -48.83472583511090903, -289.9976704382382877, -346.3890832113571605 ) ) ;
#49796=CARTESIAN_POINT ( 'NONE',  ( -38.91262770159233497, -289.5637108024761233, -347.2835405265697659 ) ) ;
#49797=CARTESIAN_POINT ( 'NONE',  ( 16.88919303119128301, -287.0189286124443129, -221.4751854650539826 ) ) ;
#49800=CARTESIAN_POINT ( 'NONE',  ( 33.30836724089176926, -295.7648982284252952, -297.7266704035982912 ) ) ;
#49801=CARTESIAN_POINT ( 'NONE',  ( -36.88358882543816009, -296.7426073036224352, -193.8543649343474158 ) ) ;
#49802=CARTESIAN_POINT ( 'NONE',  ( -80.96912369364359563, -276.7200135657021178, -329.1833617382810644 ) ) ;
#49803=CARTESIAN_POINT ( 'NONE',  ( -108.0184868496298662, -272.4489215396031341, -239.8237985079902614 ) ) ;
#49805=CARTESIAN_POINT ( 'NONE',  ( -7.727282633707822868, -293.1367174796890254, -337.8558865948379548 ) ) ;
#49806=CARTESIAN_POINT ( 'NONE',  ( 33.87899892761087273, -277.5754339134395536, -290.5467157374345675 ) ) ;
#49807=CARTESIAN_POINT ( 'NONE',  ( -91.07459420315046827, -271.4183436200209485, -219.1210316221652477 ) ) ;
#49808=CARTESIAN_POINT ( 'NONE',  ( 29.85973774946995363, -295.1521382093529269, -299.8754746736206016 ) ) ;
#49809=CARTESIAN_POINT ( 'NONE',  ( -90.62248221880751942, -296.9088923129604041, -320.7868083438918347 ) ) ;
#49810=CARTESIAN_POINT ( 'NONE',  ( -93.30409020842159862, -293.8543926363487344, -320.5623643558286631 ) ) ;
#49811=CARTESIAN_POINT ( 'NONE',  ( 98.95318904190033038, -300.3680452193383417, -193.4483179873065808 ) ) ;
#49812=CARTESIAN_POINT ( 'NONE',  ( 20.81201258752314587, -286.7571403089615956, -315.4760875844818315 ) ) ;
#49814=CARTESIAN_POINT ( 'NONE',  ( -101.1610145235557070, -273.6121516511580580, -227.2939191672174957 ) ) ;
#49815=CARTESIAN_POINT ( 'NONE',  ( -96.11986373800614558, -297.4927311286100462, -227.0131676883118530 ) ) ;
#49816=CARTESIAN_POINT ( 'NONE',  ( 23.25376937781267728, -282.9236957762963129, -225.5660749455804819 ) ) ;
#49817=CARTESIAN_POINT ( 'NONE',  ( 23.36628573990366320, -279.6116999667987102, -223.7796556094168068 ) ) ;
#49819=CARTESIAN_POINT ( 'NONE',  ( 22.43877872555829711, -281.5504122552567878, -318.7513761988834631 ) ) ;
#49820=CARTESIAN_POINT ( 'NONE',  ( 12.63207654232220101, -275.7249403157621828, -328.8071138383847369 ) ) ;
#49821=CARTESIAN_POINT ( 'NONE',  ( 36.76552342114966621, -280.1768266888805670, -288.1525459193726419 ) ) ;
#49822=CARTESIAN_POINT ( 'NONE',  ( -97.10289916224024864, -277.1748693176369329, -224.7481918372506868 ) ) ;
#49824=CARTESIAN_POINT ( 'NONE',  ( 21.96674687273048932, -273.5214148574976321, -226.7964185958797714 ) ) ;
#49825=CARTESIAN_POINT ( 'NONE',  ( -44.55529877465829713, -275.9611683749261033, -195.6574348565242758 ) ) ;
#49827=CARTESIAN_POINT ( 'NONE',  ( -44.71056285174318390, -289.9795714653202481, -195.3152822124797012 ) ) ;
#49828=CARTESIAN_POINT ( 'NONE',  ( -90.78593627599708782, -291.3195377114608391, -214.8550547389671692 ) ) ;
#49829=CARTESIAN_POINT ( 'NONE',  ( 37.79212958427492453, -277.5980497971481213, -273.9308769174308509 ) ) ;
#49830=CARTESIAN_POINT ( 'NONE',  ( 25.48235028399638580, -272.9995144579729072, -229.3960189570080104 ) ) ;
#49833=CARTESIAN_POINT ( 'NONE',  ( -111.9640761502929820, -282.4491171551121624, -278.3730152255371877 ) ) ;
#49835=CARTESIAN_POINT ( 'NONE',  ( 31.90961710675410501, -292.6706815374907933, -294.8316252812142011 ) ) ;
#49836=CARTESIAN_POINT ( 'NONE',  ( 28.10849718413521003, -286.1626175983739699, -305.5009759754066749 ) ) ;
#49839=CARTESIAN_POINT ( 'NONE',  ( -76.72950313944535594, -293.5788096785367429, -334.2464492861664098 ) ) ;
#49840=CARTESIAN_POINT ( 'NONE',  ( -37.33393347205793589, -281.5319053493707315, -346.6807339980219353 ) ) ;
#49841=CARTESIAN_POINT ( 'NONE',  ( -46.57654910983590923, -281.5332717048788140, -197.0895256130339988 ) ) ;
#49842=CARTESIAN_POINT ( 'NONE',  ( -64.42125486780727783, -286.9115405945510702, -198.6901562599271927 ) ) ;
#49843=CARTESIAN_POINT ( 'NONE',  ( 27.00534518478758983, -279.2546664424246501, -229.8467278986334748 ) ) ;
#49844=CARTESIAN_POINT ( 'NONE',  ( 35.68036566243934971, -287.5251269647072263, -268.3124598845219566 ) ) ;
#49845=CARTESIAN_POINT ( 'NONE',  ( -36.44089622264606021, -278.4659548948858401, -343.9574030452341731 ) ) ;
#49846=CARTESIAN_POINT ( 'NONE',  ( -108.3262700791548383, -279.1211240471191104, -288.1269243049661668 ) ) ;
#49847=CARTESIAN_POINT ( 'NONE',  ( -102.6283106583776714, -287.0330868518112197, -232.6266498743745217 ) ) ;
#49849=CARTESIAN_POINT ( 'NONE',  ( -57.38767208902535089, -297.6338203442297754, -195.9609744393078472 ) ) ;
#49850=CARTESIAN_POINT ( 'NONE',  ( 21.67303688889696645, -290.1617528743838079, -316.0885798910165931 ) ) ;
#49852=CARTESIAN_POINT ( 'NONE',  ( 40.64545035920995986, -283.8376638359844719, -252.5284128619064461 ) ) ;
#49854=CARTESIAN_POINT ( 'NONE',  ( 18.68676554844735094, -272.8551857226655102, -220.1763184737467043 ) ) ;
#49855=CARTESIAN_POINT ( 'NONE',  ( 10.67820443440623279, -292.8014310114523369, -329.5943707563055227 ) ) ;
#49856=CARTESIAN_POINT ( 'NONE',  ( -98.78845351809526676, -295.5121547124304584, -309.9795603880564840 ) ) ;
#49857=CARTESIAN_POINT ( 'NONE',  ( 20.04300439882612395, -288.4244788781235229, -224.1058253997332770 ) ) ;
#49858=CARTESIAN_POINT ( 'NONE',  ( 35.48653156009788745, -283.4848606421106183, -283.6240168736629244 ) ) ;
#49859=CARTESIAN_POINT ( 'NONE',  ( -9.758969124533837913, -290.1240677433547148, -341.6197963537935607 ) ) ;
#49860=CARTESIAN_POINT ( 'NONE',  ( -48.77862924457342331, -290.5099293751202367, -346.0618892339080048 ) ) ;
#49861=CARTESIAN_POINT ( 'NONE',  ( -68.59519717577731512, -285.4630320083518882, -338.5389705067708519 ) ) ;
#49862=CARTESIAN_POINT ( 'NONE',  ( -106.3444376767037198, -278.2783111592956402, -304.6515609684820447 ) ) ;
#49863=CARTESIAN_POINT ( 'NONE',  ( 34.11644967576441445, -291.9492431073694547, -295.0783180677186692 ) ) ;
#49864=CARTESIAN_POINT ( 'NONE',  ( -7.535029617025729820, -280.2655665605205968, -199.3498964331015486 ) ) ;
#49865=CARTESIAN_POINT ( 'NONE',  ( -54.51997738608783806, -275.6895067215083373, -198.1408142731350779 ) ) ;
#49866=CARTESIAN_POINT ( 'NONE',  ( 35.78497577281001440, -290.2662352645559167, -287.0191576251351080 ) ) ;
#49868=CARTESIAN_POINT ( 'NONE',  ( 30.35777514462878912, -273.3416883002064424, -235.8537990613072566 ) ) ;
#49870=CARTESIAN_POINT ( 'NONE',  ( 18.88747793414631815, -280.3985701247459019, -223.6912113599244947 ) ) ;
#49871=CARTESIAN_POINT ( 'NONE',  ( 37.24475432140723541, -276.5370697889363214, -252.8435944168766980 ) ) ;
#49873=CARTESIAN_POINT ( 'NONE',  ( -96.58539395881665257, -298.5845457343937142, -226.6871207229745551 ) ) ;
#49874=CARTESIAN_POINT ( 'NONE',  ( -90.28456718528400415, -282.8376740532990539, -326.0206415007153851 ) ) ;
#49875=CARTESIAN_POINT ( 'NONE',  ( -106.0454413714065254, -291.9472761082202510, -298.0261843923643141 ) ) ;
#49876=CARTESIAN_POINT ( 'NONE',  ( -10.64716429470371928, -275.9945981632093890, -198.9338323928342334 ) ) ;
#49877=CARTESIAN_POINT ( 'NONE',  ( -107.6311005046765956, -274.2561518344775209, -240.0161713817290945 ) ) ;
#49879=CARTESIAN_POINT ( 'NONE',  ( 11.50704648305693567, -296.3728436974096212, -327.0517554645664973 ) ) ;
#49880=CARTESIAN_POINT ( 'NONE',  ( -103.4013038288097874, -282.0833372669978303, -305.6305016335276719 ) ) ;
#49881=CARTESIAN_POINT ( 'NONE',  ( -94.69271820775296078, -290.9155900141443567, -219.0132356817496486 ) ) ;
#49882=CARTESIAN_POINT ( 'NONE',  ( 36.98965680128517164, -273.6604138287934802, -277.1945781595177891 ) ) ;
#49883=CARTESIAN_POINT ( 'NONE',  ( 25.68409957670541388, -288.5813889267474224, -227.5103852169342247 ) ) ;
#49884=EDGE_CURVE ( 'NONE', #38497, #55253, #43778, .T. ) ;
#49885=CARTESIAN_POINT ( 'NONE',  ( -97.00495677743501233, -290.0661575415214202, -227.6780694355106505 ) ) ;
#49887=CARTESIAN_POINT ( 'NONE',  ( -107.8166305711135493, -289.5053653399637028, -240.8333264887179155 ) ) ;
#49888=CARTESIAN_POINT ( 'NONE',  ( -109.6444847925146320, -290.0829406724311639, -280.6682380794902087 ) ) ;
#49890=CARTESIAN_POINT ( 'NONE',  ( 31.41640632547085232, -289.0714297820604202, -304.4487862585778544 ) ) ;
#49891=CARTESIAN_POINT ( 'NONE',  ( 16.54962570921479781, -276.5922205805587737, -319.6526059576839316 ) ) ;
#49893=CARTESIAN_POINT ( 'NONE',  ( -61.50725645781604101, -294.2790779780762591, -343.2006902315841899 ) ) ;
#49894=CARTESIAN_POINT ( 'NONE',  ( -97.95894348735140511, -284.5704908871134080, -317.6777386843335194 ) ) ;
#49895=CARTESIAN_POINT ( 'NONE',  ( -99.32974058128755246, -285.4929659885997353, -224.6310229122993576 ) ) ;
#49896=CARTESIAN_POINT ( 'NONE',  ( 25.57940460067867861, -282.3954333990724308, -307.5153564327474101 ) ) ;
#49897=CARTESIAN_POINT ( 'NONE',  ( 167.9348045515096999, 232.6400991984046982, -192.7129745902395541 ) ) ;
#49898=CARTESIAN_POINT ( 'NONE',  ( 166.7220858323138657, 232.6500979171330243, -192.0954861747825362 ) ) ;
#49899=CARTESIAN_POINT ( 'NONE',  ( 201.2091912597866781, 293.0223957429525399, -68.25549348882485390 ) ) ;
#49900=CARTESIAN_POINT ( 'NONE',  ( -109.2866109036451547, -271.9277654570573191, -256.8038092756640935 ) ) ;
#49901=CARTESIAN_POINT ( 'NONE',  ( -40.77571630126477942, -272.9284093343463837, -197.0825670178670634 ) ) ;
#49902=CARTESIAN_POINT ( 'NONE',  ( -0.7409784574130733326, -294.0870274742118795, -338.0510532825337577 ) ) ;
#49903=CARTESIAN_POINT ( 'NONE',  ( 194.1843140057649180, 275.6304509567530090, -124.2126573568886130 ) ) ;
#49904=CARTESIAN_POINT ( 'NONE',  ( -46.80330380301038673, -272.6192283555371887, -194.4415794704493123 ) ) ;
#49905=CARTESIAN_POINT ( 'NONE',  ( -94.58089565245009567, -299.0716829612376841, -223.0704147883828909 ) ) ;
#49906=CARTESIAN_POINT ( 'NONE',  ( 6.149853404731024931, -289.7634432556220645, -329.6675105043229905 ) ) ;
#49907=CARTESIAN_POINT ( 'NONE',  ( -93.68620571708281375, -292.2945742797382991, -223.4424461779046851 ) ) ;
#49909=CARTESIAN_POINT ( 'NONE',  ( -108.1533424280992790, -297.1136974343089037, -300.1386756128952129 ) ) ;
#49910=CARTESIAN_POINT ( 'NONE',  ( -5.777737175144225468, -286.9710166889316838, -204.4557096529882756 ) ) ;
#49911=CARTESIAN_POINT ( 'NONE',  ( -0.7739967851248829023, -295.3819980031690875, -337.9552737183033742 ) ) ;
#49912=CARTESIAN_POINT ( 'NONE',  ( -98.22191719684298050, -296.4160370038868564, -317.4049919001111562 ) ) ;
#49913=CARTESIAN_POINT ( 'NONE',  ( 35.62126243195009323, -293.6881613454568765, -268.0360160606145996 ) ) ;
#49915=CARTESIAN_POINT ( 'NONE',  ( -94.94605581947607220, -275.1441773710411667, -221.4427998460582216 ) ) ;
#49917=CARTESIAN_POINT ( 'NONE',  ( -96.76589954008809968, -278.7170006614438194, -221.4704843348012560 ) ) ;
#49918=CARTESIAN_POINT ( 'NONE',  ( 12.09740312572577459, -273.1529084986812563, -215.4998132229447378 ) ) ;
#49919=CARTESIAN_POINT ( 'NONE',  ( 31.48700090851100342, -276.8274603059280707, -295.5289102498280727 ) ) ;
#49920=CARTESIAN_POINT ( 'NONE',  ( 37.49020875899221750, -277.1441014553167861, -257.0899434384185724 ) ) ;
#49921=CARTESIAN_POINT ( 'NONE',  ( 37.10662818347357472, -273.4222446961183550, -258.6221591936090931 ) ) ;
#49922=CARTESIAN_POINT ( 'NONE',  ( -93.69746017186588460, -297.8628762267681509, -223.7807039619924581 ) ) ;
#49923=CARTESIAN_POINT ( 'NONE',  ( -108.7422698158706709, -295.3606841369601170, -252.4957229784031085 ) ) ;
#49925=CARTESIAN_POINT ( 'NONE',  ( -110.4931335231892859, -279.3465685677120405, -246.3509518847648394 ) ) ;
#49926=CARTESIAN_POINT ( 'NONE',  ( 18.30978838515730089, -276.3905736382098439, -317.6042320923178295 ) ) ;
#49927=CARTESIAN_POINT ( 'NONE',  ( -29.49674674230796256, -284.8343792380504169, -194.2575373921601454 ) ) ;
#49928=CARTESIAN_POINT ( 'NONE',  ( -110.4982369779130238, -274.7645059412130308, -253.8347218290428771 ) ) ;
#49929=CARTESIAN_POINT ( 'NONE',  ( 82.67722570198282028, -297.3296337185574316, -196.5151116418807931 ) ) ;
#49930=CARTESIAN_POINT ( 'NONE',  ( 24.36907679217138423, -287.2914998494832162, -309.6597405889123706 ) ) ;
#49931=CARTESIAN_POINT ( 'NONE',  ( -38.34538218574085278, -278.2792632068584453, -196.3420145611505632 ) ) ;
#49932=CARTESIAN_POINT ( 'NONE',  ( -14.10575345053863572, -278.9341216763961029, -200.4827074408945577 ) ) ;
#49934=CARTESIAN_POINT ( 'NONE',  ( -93.97195694407641042, -285.8698452214187000, -319.5537570489542532 ) ) ;
#49935=CARTESIAN_POINT ( 'NONE',  ( -59.29924859845507257, -278.5479144188467444, -340.3967986692132399 ) ) ;
#49936=B_SPLINE_CURVE_WITH_KNOTS ( 'NONE', 3,
 ( #56300, #20776, #393, #79484, #92727, #49187, #72373, #13682, #93203, #7490, #70974, #27899, #6107, #36375, #71444, #65288, #85630, #29282, #6581, #49648, #50107, #28355, #86087, #79002, #5482, #68936, #26779, #77920, #11158, #55200, #13062, #84986, #19664, #56621, #85472, #12577, #34354, #70356, #40472, #49023, #76502, #4067, #63259, #41898, #83579, #12095, #11626, #92090, #48532, #76030, #54702, #32937, #77433, #34816, #47117, #26305, #18741, #55665, #84055, #19202, #40019, #27725, #41424, #47600, #76966, #61829, #90662, #25822, #27247, #62791, #91626, #69389, #56133, #4522, #69862, #33398, #62297, #33882, #92554, #91138, #48062, #5000, #40942, #84517, #20141, #70812, #5944, #63729, #93039, #35758, #78838, #50888, #7787, #58472, #28652, #13520, #232, #85923, #72668, #21074, #51336, #13984, #93499, #37143, #57543, #65595, #14462, #708, #80230, #71760, #29593, #86386, #66050, #49945, #79769, #36673, #21537, #7331, #29112, #57084, #1163, #42845, #50420, #30046, #79324, #87316, #43319, #22464, #15366, #6885, #44227, #72215, #36211, #73137, #8262, #58927, #65130, #58008, #64671, #78379, #86863, #22018, #14912, #20619, #49489, #42368, #43767, #71280, #6407, #64209, #35282, #28196, #23408, #9169, #17234, #10575, #44700, #32375, #31443, #8712, #9649, #45613, #1619, #30502, #51797, #38533, #81610, #24801, #67437, #46096, #15842, #2564, #53686, #80689, #2095, #82554, #31901, #60332, #3482, #87777, #53198, #45151, #23861, #3015, #89169, #24321, #73601, #75001, #17702, #59397, #52727, #52275, #38979, #82076, #22927, #88251, #37589, #10113, #75455, #66500, #66956, #46555, #39438, #81154, #16298, #38047, #68354, #67892, #74050, #16759, #30985, #59873, #88713, #60793, #89631, #74514, #68831, #55561, #90110, #83952, #3960, #25262, #33769, #54139, #41308, #4885, #19102, #32834, #83008, #61724, #62191, #76399, #11986, #39911, #11522, #25714, #91515, #5835, #47957, #76861, #61275, #69286, #26671, #40835, #40369, #84409, #41793, #27135, #91021, #47491, #69754, #62681, #55084, #56019, #19557, #47013, #18160, #75916, #48423, #90556, #54598, #11041, #77328, #12461, #83469, #70245, #34245, #26190, #18625, #4415, #5379, #33293, #91982, #63151, #20026, #84875, #48903, #77805, #12955, #70704, #43661, #64090, #35650, #56507, #6300, #78730, #120, #92446, #35168, #595, #21906, #22353, #92930, #28091, #13873, #51227, #86275, #56977, #58365, #87205, #73017, #27609, #29477, #72111, #57434, #71641, #42725, #63621, #93391, #79665, #64566, #85815, #6774, #7227, #20966, #20514, #49382, #28543, #85365, #36101, #78275, #13413, #65020, #42257, #49833, #21428, #29003, #50301, #79207, #80115, #15254, #57888, #14350, #44115, #43209, #86744, #50779, #14806, #72556, #7678, #71171, #65477, #36563, #34707, #38868, #88599, #9995, #87663, #30389, #81493, #73488, #59281, #1503, #9052, #53565, #66387, #60678, #16184, #74885, #51682, #89054, #37029, #15724, #29933, #74396, #89518, #46437, #81040, #44585, #16640, #45035, #73937, #1054, #67774, #45494, #30865, #37930, #66839, #65943, #1973, #53080, #23748, #52611, #8600, #2450, #58818, #59759, #37477, #22812, #9525, #82440, #88126, #80570, #38411, #23285, #52158, #67320, #31328, #60215, #24203, #2901, #81958, #17114, #45980, #31784, #24681, #17588, #8146, #54958, #46898, #33650, #75799, #12340, #10923, #19445, #41188, #62070, #77212, #61158, #3843, #83835, #32725, #68713, #76280, #27021, #39790, #34132, #83353, #48311, #25149, #62558, #18989, #19912, #33181, #90904, #75340, #70126, #10456, #61612, #5263, #91400, #55910, #63036, #11406, #90444, #47841, #76743, #69174, #91867, #26555, #89994, #68240, #54023, #26071, #82890, #18046, #39322, #11871, #4303, #84762, #40723, #3363, #40258, #32251, #25601, #69639, #54484, #18503, #55443, #47365, #4767, #84295, #59596, #44427, #23113, #2291, #37777, #30696, #43953, #74240, #24047, #52462, #51068, #87500, #52922, #9360, #22649, #16948, #45339, #36872, #87050, #38244, #51521, #8444, #16483, #9841, #72850, #31629, #88446, #7978, #8899, #44882, #896, #29779, #79955, #66683, #80883, #81801, #1810, #67158, #15093, #23595, #45812, #65787, #1345, #74721, #31174, #81336, #2749, #22199, #60060, #73333, #51996, #88898, #38714, #67621, #58658, #80408, #15555, #37323, #16031, #66231, #30228, #59119, #87960, #73784, #82279, #33021, #48146, #5088, #39624, #84137, #19287, #60520, #39167, #10766, #41022, #90747, #3204, #90295, #69945, #53394, #89356, #47685, #76116, #11249, #68079, #54787, #24512, #83199, #32088, #17431, #61911, #46280, #40561, #4150, #18347, #60989, #75184, #89837, #61464, #75643, #40103, #24998, #68548, #53870, #25905, #76586, #4607, #3687, #10297, #47202, #69019, #82736, #17888, #46740, #32572, #25447, #77048, #54324, #11709, #83666, #69475, #26395, #18830, #33480, #62383, #91228, #12178 ),
 .UNSPECIFIED., .F., .F.,
 ( 4, 1, 1, 1, 2, 2, 2, 2, 2, 2, 2, 2, 2, 2, 2, 2, 2, 2, 2, 2, 2, 2, 2, 2, 2, 2, 2, 2, 2, 2, 2, 2, 2, 2, 2, 2, 2, 2, 2, 2, 2, 2, 2, 2, 2, 2, 2, 2, 2, 2, 2, 2, 2, 2, 2, 2, 2, 2, 2, 2, 2, 2, 2, 2, 2, 2, 2, 2, 2, 2, 2, 2, 2, 2, 2, 2, 2, 2, 2, 2, 2, 2, 2, 2, 2, 2, 2, 2, 2, 2, 2, 2, 2, 2, 2, 2, 2, 2, 2, 2, 2, 2, 2, 2, 2, 2, 2, 2, 2, 2, 2, 2, 2, 2, 2, 2, 2, 2, 2, 2, 2, 2, 2, 2, 2, 2, 2, 2, 2, 2, 2, 2, 2, 2, 2, 2, 2, 2, 2, 2, 2, 2, 2, 2, 2, 2, 2, 2, 2, 2, 2, 2, 2, 2, 2, 2, 2, 2, 2, 2, 2, 2, 2, 2, 2, 2, 2, 2, 2, 2, 2, 2, 2, 2, 2, 2, 2, 2, 2, 2, 2, 2, 2, 2, 2, 2, 2, 2, 2, 2, 2, 2, 2, 2, 2, 2, 2, 2, 2, 2, 2, 2, 2, 2, 2, 2, 2, 2, 2, 2, 2, 2, 2, 2, 2, 2, 2, 2, 2, 2, 2, 2, 2, 2, 2, 2, 2, 2, 2, 2, 2, 2, 2, 2, 2, 2, 2, 2, 2, 2, 2, 2, 2, 2, 2, 2, 2, 2, 2, 2, 2, 2, 2, 2, 2, 2, 2, 2, 2, 2, 2, 2, 2, 2, 2, 2, 2, 2, 2, 2, 2, 2, 2, 2, 2, 2, 2, 2, 2, 2, 2, 2, 2, 2, 2, 2, 2, 2, 2, 2, 2, 2, 2, 2, 2, 2, 2, 2, 2, 2, 4 ),
 ( -0.05114148247438684430, -0.02298081116268822083, -0.008900475506838909090, -0.001860307678914256690, -0.0001002657219330849170, 0.0007797552565574905614, 0.001659776235048066040, 0.005179860149010367953, 0.008699944062972676806, 0.01222002797693497872, 0.01398006993391614355, 0.01574011189089730839, 0.01926019580485965194, 0.02278027971882199548, 0.02630036363278432515, 0.02806040558976548999, 0.02982044754674665482, 0.03334053146070899837, 0.03686061537467134192, 0.04038069928863367158, 0.04214074124561486417, 0.04390078320259605676, 0.04742086711655842807, 0.05094095103052078549, 0.05446103494448314292, 0.05622107690146430775, 0.05798111885844545871, 0.06150120277240774674, 0.06502128668637005560, 0.06854137060033232975, 0.07030141255731350847, 0.07206145451429465942, 0.07558153842825710012, 0.07910162234221954081, 0.08262170625618195374, 0.08438174821316321572, 0.08614179017014442219, 0.08966187408410689064, 0.09318195799806935908, 0.09670204191203182753, 0.09846208386901306175, 0.1002221258259942960, 0.1037422097399567644, 0.1072622936539192606, 0.1107823775678817291, 0.1143024614818441975, 0.1178225453958066660, 0.1213426293097691622, 0.1248627132237316306, 0.1283827971376941268, 0.1301428390946753610, 0.1319028810516565953, 0.1354229649656189804, 0.1389430488795813934, 0.1424631327935438063, 0.1442231747505249573, 0.1459832167075061360, 0.1495033006214684657, 0.1530233845354307953, 0.1565434684493930972, 0.1583035104063742760, 0.1600635523633553992, 0.1635836362773177288, 0.1671037201912800307, 0.1706238041052423327, 0.1723838460622234836, 0.1741438880192046346, 0.1776639719331669642, 0.1811840558471292661, 0.1847041397610916236, 0.1864641817180728023, 0.1882242236750539255, 0.1917443075890162829, 0.1952643915029785848, 0.1987844754169409145, 0.2005445173739221210, 0.2023045593309032719, 0.2058246432448655738, 0.2093447271588279313, 0.2128648110727902332, 0.2146248530297713841, 0.2163848949867525906, 0.2199049789007148925, 0.2234250628146771944, 0.2269451467286395518, 0.2287051886856207028, 0.2304652306426018538, 0.2339853145565642112, 0.2375053984705265131, 0.2410254823844888705, 0.2427855243414700215, 0.2445455662984512279, 0.2480656502124134744, 0.2515857341263758040, 0.2551058180403380504, 0.2568658599973192014, 0.2586259019543003523, 0.2621459858682626543, 0.2656660697822250117, 0.2691861536961873691, 0.2709461956531685756, 0.2727062376101497820, 0.2762263215241121950, 0.2797464054380744969, 0.2832664893520369098, 0.2850265313090181718, 0.2867865732659993228, 0.2903066571799617912, 0.2938267410939241486, 0.2973468250078865061, 0.2991068669648677680, 0.3008669089218489745, 0.3043869928358113319, 0.3079070767497736894, 0.3114271606637361023, 0.3131872026207173088, 0.3149472445776985152, 0.3184673284916609282, 0.3219874124056232856, 0.3255074963195856430, 0.3272675382765669050, 0.3290275802335480559, 0.3325476641475105244, 0.3360677480614729373, 0.3395878319754353503, 0.3413478739324165567, 0.3431079158893978187, 0.3466279998033601761, 0.3501480837173225336, 0.3536681676312848910, 0.3571882515452473039, 0.3607083354592097169, 0.3642284193731720188, 0.3677485032871344317, 0.3712685872010967891, 0.3730286291580779956, 0.3747886711150591466, 0.3783087550290215040, 0.3818288389429838059, 0.3853489228569461633, 0.3871089648139272588, 0.3888690067709084652, 0.3923890906848707671, 0.3959091745988330691, 0.3994292585127954265, 0.4011893004697765774, 0.4029493424267577839, 0.4064694263407201413, 0.4099895102546823877, 0.4135095941686447452, 0.4152696361256259516, 0.4170296780826071026, 0.4205497619965694045, 0.4240698459105317619, 0.4275899298244940083, 0.4293499717814752703, 0.4311100137384563658, 0.4346300976524188342, 0.4381501815663812471, 0.4416702654803436046, 0.4434303074373248665, 0.4451903493943059620, 0.4487104333082684304, 0.4522305172222308989, 0.4557506011361933118, 0.4575106430931744073, 0.4592706850501556137, 0.4627907689641180267, 0.4663108528780804396, 0.4698309367920429636, 0.4715909787490241700, 0.4733510207060054875, 0.4768711046199679005, 0.4803911885339304244, 0.4839112724478930594, 0.4856713144048742659, 0.4874313563618555833, 0.4909514402758181073, 0.4944715241897805202, 0.4979916081037431552, 0.4997516500607243617, 0.5015116920177056237, 0.5050317759316681476, 0.5085518598456305606, 0.5120719437595931955, 0.5138319857165745130, 0.5155920276735557195, 0.5191121115875182435, 0.5226321955014807674, 0.5261522794154432914, 0.5279123213724246089, 0.5296723633294058153, 0.5331924472433682283, 0.5367125311573306412, 0.5402326150712931652, 0.5419926570282743716, 0.5437526989852555781, 0.5472727828992179910, 0.5507928668131805150, 0.5543129507271429279, 0.5560729926841241344, 0.5578330346411054519, 0.5613531185550678648, 0.5648732024690302778, 0.5683932863829926907, 0.5701533283399738972, 0.5719133702969553257, 0.5754334542109176276, 0.5789535381248800405, 0.5824736220388425645, 0.5842336639958237710, 0.5859937059528050884, 0.5895137898667675014, 0.5930338737807299143, 0.5965539576946923273, 0.6000740416086547402, 0.6035941255226172641, 0.6071142094365796771, 0.6106342933505419790, 0.6141543772645045030, 0.6176744611784669159, 0.6211945450924293288, 0.6247146290063917418, 0.6282347129203541547, 0.6299947548773354722, 0.6317547968343166787, 0.6352748807482792026, 0.6387949646622416155, 0.6423150485762039175, 0.6440750905331852350, 0.6458351324901665524, 0.6493552164041290764, 0.6528753003180916004, 0.6563953842320541243, 0.6581554261890353308, 0.6599154681460166483, 0.6634355520599792833, 0.6669556359739419182, 0.6704757198879045532, 0.6722357618448857597, 0.6739958038018670772, 0.6775158877158296011, 0.6810359716297923471, 0.6845560555437549821, 0.6863160975007362996, 0.6880761394577177281, 0.6915962233716802521, 0.6951163072856428871, 0.6986363911996055220, 0.7003964331565868395, 0.7021564751135682680, 0.7056765590275310140, 0.7091966429414936490, 0.7127167268554563950, 0.7144767688124378235, 0.7162368107694191410, 0.7197568946833818870, 0.7232769785973446330, 0.7267970625113073790, 0.7303171464252701250, 0.7338372303392328710, 0.7373573142531956170, 0.7408773981671583631, 0.7426374401241396805, 0.7443974820811209980, 0.7479175659950836330, 0.7514376499090462680, 0.7549577338230089030, 0.7567177757799902205, 0.7584778177369715380, 0.7619979016509341729, 0.7655179855648969189, 0.7690380694788595539, 0.7707981114358408714, 0.7725581533928222999, 0.7760782373067848239, 0.7795983212207474589, 0.7831184051347100938, 0.7848784470916913003, 0.7866384890486726178, 0.7901585729626353638, 0.7936786568765978878, 0.7971987407905605227, 0.7989587827475419513, 0.8007188247045232687, 0.8042389086184859037, 0.8077589925324485387, 0.8112790764464110627, 0.8130391184033924912, 0.8147991603603738087, 0.8183192442743365547, 0.8218393281882991896, 0.8253594121022617136, 0.8271194540592430311, 0.8288794960162242376, 0.8323995799301868725, 0.8359196638441495075, 0.8394397477581122535, 0.8429598316720747775, 0.8464799155860374125, 0.8499999995000000474 ),
 .UNSPECIFIED. ) ;
#49938=CARTESIAN_POINT ( 'NONE',  ( -98.84297425056954012, -276.1918105779139978, -315.0102310916517467 ) ) ;
#49940=CARTESIAN_POINT ( 'NONE',  ( -40.78803848670462173, -274.6592142832270724, -197.2906976340829885 ) ) ;
#49941=CARTESIAN_POINT ( 'NONE',  ( 32.60874082869640489, -283.1933631683393742, -242.7061953222809620 ) ) ;
#49944=CARTESIAN_POINT ( 'NONE',  ( -26.32980674612250382, -290.8331944710387233, -345.1143948346768866 ) ) ;
#49945=CARTESIAN_POINT ( 'NONE',  ( 37.58299951730145949, -291.4960744939204460, -266.0064704915159268 ) ) ;
#49946=CARTESIAN_POINT ( 'NONE',  ( 82.17440492340898572, -297.5479941798179766, -195.4018648718562758 ) ) ;
#49947=CARTESIAN_POINT ( 'NONE',  ( 23.46973980794102133, -273.6666490244173815, -229.0685454680651958 ) ) ;
#49948=CARTESIAN_POINT ( 'NONE',  ( 28.59433252085374377, -291.2356437154830360, -236.2538595750842205 ) ) ;
#49949=CARTESIAN_POINT ( 'NONE',  ( 10.80643407470098794, -61.58976173765800155, -353.1561788127373802 ) ) ;
#49951=CARTESIAN_POINT ( 'NONE',  ( -59.84147477128698256, -287.8183871765951949, -343.2752311041638222 ) ) ;
#49952=CARTESIAN_POINT ( 'NONE',  ( -64.32915313783280453, -285.0104479084794207, -339.0496744937643712 ) ) ;
#49953=CARTESIAN_POINT ( 'NONE',  ( -2.665074207940166140, -284.7440948665608857, -202.7336474404863225 ) ) ;
#49954=CARTESIAN_POINT ( 'NONE',  ( -40.23953651559801870, -284.5145646323277333, -343.8932705592785055 ) ) ;
#49955=CARTESIAN_POINT ( 'NONE',  ( -105.3602928414461957, -284.9936877729901994, -297.4447114687678209 ) ) ;
#49956=CARTESIAN_POINT ( 'NONE',  ( -44.76074966074679651, -293.9387174026987850, -195.3202298937241039 ) ) ;
#49957=CARTESIAN_POINT ( 'NONE',  ( 31.69400916265432144, -274.0315022388318766, -301.0756916892908635 ) ) ;
#49958=CARTESIAN_POINT ( 'NONE',  ( 18.07142704441768544, -275.1528975929713283, -216.8511909310712440 ) ) ;
#49959=CARTESIAN_POINT ( 'NONE',  ( -111.7496423533197145, -288.7995213023934298, -257.2168289779902466 ) ) ;
#49960=CARTESIAN_POINT ( 'NONE',  ( -96.14919039427111613, -277.8822763525339496, -320.0873948776813904 ) ) ;
#49961=CARTESIAN_POINT ( 'NONE',  ( 37.17494982320157249, -295.4651766209661901, -265.1775562567756310 ) ) ;
#49963=CARTESIAN_POINT ( 'NONE',  ( 10.59707575819634329, -295.1948066931273615, -210.1954327657594490 ) ) ;
#49964=CARTESIAN_POINT ( 'NONE',  ( -93.62202789313710127, -283.9036784939293057, -223.0983611230452084 ) ) ;
#49965=CARTESIAN_POINT ( 'NONE',  ( -36.74227282106746628, -278.0595291278528975, -195.3508019111592091 ) ) ;
#49966=CARTESIAN_POINT ( 'NONE',  ( -68.54269788882368175, -272.1294591379420922, -200.7106174634450042 ) ) ;
#49967=CARTESIAN_POINT ( 'NONE',  ( -59.23341496180492527, -276.6917244709753163, -340.1081285966567975 ) ) ;
#49968=CARTESIAN_POINT ( 'NONE',  ( 7.078905814450073386, -294.1898900028027128, -211.5604588173541174 ) ) ;
#49969=CARTESIAN_POINT ( 'NONE',  ( 32.57499248578534434, -294.7813057824154725, -292.1570933492282052 ) ) ;
#49970=CARTESIAN_POINT ( 'NONE',  ( -70.57839402521152294, -296.7963447966814101, -339.2857686870148655 ) ) ;
#49971=CARTESIAN_POINT ( 'NONE',  ( -110.0501054498872691, -296.4786513967191013, -263.2975445926482507 ) ) ;
#49972=CARTESIAN_POINT ( 'NONE',  ( -26.15201131581959970, -290.9099957412431081, -344.5741468933361489 ) ) ;
#49973=CARTESIAN_POINT ( 'NONE',  ( -110.6848982627649178, -284.4235528446827743, -293.8518830798702197 ) ) ;
#49974=CARTESIAN_POINT ( 'NONE',  ( -94.14446629654599974, -271.3817415821985719, -220.2237941849799654 ) ) ;
#49975=CARTESIAN_POINT ( 'NONE',  ( 23.86272689839336891, -286.7623067945394268, -223.6167196894971312 ) ) ;
#49976=CARTESIAN_POINT ( 'NONE',  ( -107.8087820482681565, -280.2099084882878515, -295.1396067773449090 ) ) ;
#49977=CARTESIAN_POINT ( 'NONE',  ( -98.29628346355481483, -284.1726373679227891, -229.7662018160411606 ) ) ;
#49978=CARTESIAN_POINT ( 'NONE',  ( -107.9904147739487712, -288.2239917004074528, -295.6898193521115559 ) ) ;
#49979=CARTESIAN_POINT ( 'NONE',  ( -51.00049622308160480, -154.6998088915060237, -359.8797964913271130 ) ) ;
#49980=CARTESIAN_POINT ( 'NONE',  ( 16.02369730450794094, -286.3423523712069141, -220.4415237970370356 ) ) ;
#49981=CARTESIAN_POINT ( 'NONE',  ( 23.22468854747723910, -283.1256281732290745, -317.5473166582940507 ) ) ;
#49982=CARTESIAN_POINT ( 'NONE',  ( -114.1331516043878480, -289.6361445254684668, -268.3488820958181122 ) ) ;
#49983=CARTESIAN_POINT ( 'NONE',  ( -73.40519736204895196, -281.1821234153238152, -203.2205836637277514 ) ) ;
#49984=CARTESIAN_POINT ( 'NONE',  ( -110.8679762718638955, -280.1341592762694859, -249.2143690663019981 ) ) ;
#49985=CARTESIAN_POINT ( 'NONE',  ( -1.964219354252200178, -280.3680026367551932, -206.5063307022557240 ) ) ;
#49986=CARTESIAN_POINT ( 'NONE',  ( 21.12850565075724774, -276.8912531468064344, -223.9393622968399598 ) ) ;
#49987=CARTESIAN_POINT ( 'NONE',  ( 6.614001572301820175, -294.4729801561877025, -333.6470975303669775 ) ) ;
#49988=CARTESIAN_POINT ( 'NONE',  ( -61.81761491615411330, -287.3919497729942805, -340.8790334142558436 ) ) ;
#49989=CARTESIAN_POINT ( 'NONE',  ( -68.02551635220173409, -293.2561245674103247, -200.5977489755723582 ) ) ;
#49990=CARTESIAN_POINT ( 'NONE',  ( -88.72829054802704718, -294.7142789891280472, -322.7167368490790409 ) ) ;
#49992=CARTESIAN_POINT ( 'NONE',  ( -5.393159943599763473, -284.5487333360299544, -337.6105856441724313 ) ) ;
#49993=CARTESIAN_POINT ( 'NONE',  ( -106.7255447496959846, -296.5227493353484647, -247.4419006604565823 ) ) ;
#49994=CARTESIAN_POINT ( 'NONE',  ( -22.26805625430534974, -293.3203818394849804, -195.1120797738107910 ) ) ;
#49995=CARTESIAN_POINT ( 'NONE',  ( 35.78914642240709298, -282.1800118415428074, -268.5728174589726791 ) ) ;
#49996=CARTESIAN_POINT ( 'NONE',  ( -60.78781625148388912, -272.8140667961619670, -197.2091506282590956 ) ) ;
#49997=CARTESIAN_POINT ( 'NONE',  ( -41.74641657612756518, -289.7576548684417617, -347.1461356101472120 ) ) ;
#49998=CARTESIAN_POINT ( 'NONE',  ( -97.08527888746390033, -282.0590682803995151, -316.9552193414020280 ) ) ;
#50000=CARTESIAN_POINT ( 'NONE',  ( -88.63855353245243407, -291.6885423064632619, -212.9644532514443540 ) ) ;
#50001=CARTESIAN_POINT ( 'NONE',  ( 16.02931784716777486, -288.6026706362052323, -320.2710579388211727 ) ) ;
#50004=CARTESIAN_POINT ( 'NONE',  ( 196.6421184343808193, 281.7221770927952207, -110.2479207600687516 ) ) ;
#50006=CARTESIAN_POINT ( 'NONE',  ( -85.28047601435909542, -270.9094976428775681, -210.1954327657594206 ) ) ;
#50007=CARTESIAN_POINT ( 'NONE',  ( -87.63422226383934799, -278.5255360678094689, -217.1567198283532889 ) ) ;
#50009=CARTESIAN_POINT ( 'NONE',  ( -74.65131410698072045, -278.4637608769353960, -207.1979521230794887 ) ) ;
#50010=CARTESIAN_POINT ( 'NONE',  ( 22.74451162792970393, -274.5739322906576945, -222.2216988036958014 ) ) ;
#50011=CARTESIAN_POINT ( 'NONE',  ( -110.3740690499103749, -272.8271011984412553, -283.8530902933177913 ) ) ;
#50012=CARTESIAN_POINT ( 'NONE',  ( -94.50880747682556660, -277.8191335602747927, -219.6607419386456570 ) ) ;
#50013=CARTESIAN_POINT ( 'NONE',  ( -5.350386419023300810, -280.6493188996844879, -337.8170228336247760 ) ) ;
#50014=CARTESIAN_POINT ( 'NONE',  ( -112.3922847719415188, -298.4640266242891471, -258.3880479038497242 ) ) ;
#50015=CARTESIAN_POINT ( 'NONE',  ( 22.98734806831856048, -294.6185109508961659, -311.6611798477420621 ) ) ;
#50017=CARTESIAN_POINT ( 'NONE',  ( -98.53048209343150177, -288.6754195420510314, -311.0924680925500638 ) ) ;
#50018=CARTESIAN_POINT ( 'NONE',  ( -1.356548821269418781, -275.1681274408801414, -202.4024417720908673 ) ) ;
#50019=CARTESIAN_POINT ( 'NONE',  ( -76.56422738799662397, -273.5111542454246205, -208.7933231922218056 ) ) ;
#50024=CARTESIAN_POINT ( 'NONE',  ( 19.90883224788790073, -281.9876375116658096, -224.5724445204919277 ) ) ;
#50025=CARTESIAN_POINT ( 'NONE',  ( -53.56626286476127774, -281.6070426620511284, -196.0729217802764310 ) ) ;
#50026=CARTESIAN_POINT ( 'NONE',  ( -107.9913014393528812, -283.3563270936316485, -289.6968913261640068 ) ) ;
#50027=CARTESIAN_POINT ( 'NONE',  ( -43.88315029685729485, -281.8291573199855975, -196.3636013321710436 ) ) ;
#50028=CARTESIAN_POINT ( 'NONE',  ( 32.72703048520246227, -273.7300393484001120, -247.3696343110754867 ) ) ;
#50031=CARTESIAN_POINT ( 'NONE',  ( -51.27328725340623805, -278.0287571111343823, -345.9261211268482725 ) ) ;
#50035=CARTESIAN_POINT ( 'NONE',  ( -33.12502947872636838, -284.9792081295841513, -345.6111072953592043 ) ) ;
#50036=CARTESIAN_POINT ( 'NONE',  ( 30.98283435409080511, -292.4007101989516286, -244.2008482125474131 ) ) ;
#50037=CARTESIAN_POINT ( 'NONE',  ( 38.98833348891655248, -287.0229320956844390, -280.1184906954568987 ) ) ;
#50038=CARTESIAN_POINT ( 'NONE',  ( -100.4619602754840741, -283.3184626201401670, -231.6137203340301483 ) ) ;
#50039=CARTESIAN_POINT ( 'NONE',  ( -90.07250555346972476, -283.8639279031973501, -218.9573483226625683 ) ) ;
#50040=CARTESIAN_POINT ( 'NONE',  ( 8.591538043416290904, -286.6526909978351796, -328.3965523477402257 ) ) ;
#50041=CARTESIAN_POINT ( 'NONE',  ( 22.91950354912111010, -283.3380699810228407, -312.2624047959108111 ) ) ;
#50042=CARTESIAN_POINT ( 'NONE',  ( -38.30548008206496036, -272.0399123560097223, -195.3673063639620864 ) ) ;
#50043=CARTESIAN_POINT ( 'NONE',  ( -69.43711815090962602, -284.0367239618503277, -201.2359448963899808 ) ) ;
#50044=CARTESIAN_POINT ( 'NONE',  ( -94.05208249591784408, -297.8715440663210074, -319.4420020705679804 ) ) ;
#50045=CARTESIAN_POINT ( 'NONE',  ( -18.61358390961857268, -284.2925103463169876, -197.5111273657321078 ) ) ;
#50046=CARTESIAN_POINT ( 'NONE',  ( -110.5147438345516093, -279.4537126266886276, -273.3800784291963737 ) ) ;
#50047=CARTESIAN_POINT ( 'NONE',  ( 12.99968803966445208, -288.7529821462077280, -214.4721992003050275 ) ) ;
#50052=CARTESIAN_POINT ( 'NONE',  ( 36.90562894240503766, -295.2935817163242405, -256.3379825907792906 ) ) ;
#50053=CARTESIAN_POINT ( 'NONE',  ( -111.0943360317898936, -276.7268931420227887, -256.7394679982444927 ) ) ;
#50054=CARTESIAN_POINT ( 'NONE',  ( -112.7644876348830110, -289.9341866814194191, -255.6105936382482184 ) ) ;
#50055=CARTESIAN_POINT ( 'NONE',  ( -56.02530817874509950, -293.6965266030794623, -341.8099003453828004 ) ) ;
#50056=CARTESIAN_POINT ( 'NONE',  ( -69.94408142513989901, -278.2982957920120839, -204.4811941811498173 ) ) ;
#50057=CARTESIAN_POINT ( 'NONE',  ( -72.22481840170092937, -295.7252059208834680, -204.8178063481725815 ) ) ;
#50058=CARTESIAN_POINT ( 'NONE',  ( -98.72057099681400416, -292.4252351299080033, -229.8473941049495863 ) ) ;
#50059=CARTESIAN_POINT ( 'NONE',  ( -4.771743288812468897, -279.1233781216988064, -337.9199732462171255 ) ) ;
#50060=CARTESIAN_POINT ( 'NONE',  ( -92.21201882117370019, -294.2990334148379930, -323.3889962992760161 ) ) ;
#50061=CARTESIAN_POINT ( 'NONE',  ( -80.86302828035412915, -291.2537262982968400, -330.0261598545494053 ) ) ;
#50062=CARTESIAN_POINT ( 'NONE',  ( -40.56667927183256950, -290.2520131233092684, -194.4299062573696517 ) ) ;
#50063=CARTESIAN_POINT ( 'NONE',  ( -15.66086487428782981, -290.1914726447376438, -340.7373172693251604 ) ) ;
#50065=CARTESIAN_POINT ( 'NONE',  ( -108.5051090615654488, -291.1314463266905932, -287.3426066244903723 ) ) ;
#50067=CARTESIAN_POINT ( 'NONE',  ( -98.04307686021779489, -292.3841646566975214, -223.6135392585177897 ) ) ;
#50068=CARTESIAN_POINT ( 'NONE',  ( 20.71985670166316140, -278.9125068340608777, -222.3271464094816565 ) ) ;
#50069=CARTESIAN_POINT ( 'NONE',  ( -108.9387314423978665, -290.3634189425060868, -284.6681278710166794 ) ) ;
#50070=CARTESIAN_POINT ( 'NONE',  ( -56.55548076943339453, -280.1444690109732392, -195.7636948748492500 ) ) ;
#50072=CARTESIAN_POINT ( 'NONE',  ( 38.12398136993925135, -281.4088717274607347, -285.5491134939606468 ) ) ;
#50073=CARTESIAN_POINT ( 'NONE',  ( 33.74412471680724934, -285.2428112635882371, -246.4486493887201277 ) ) ;
#50074=DIRECTION ( 'NONE',  ( 0.000000000000000000, 0.000000000000000000, 1.000000000000000000 ) ) ;
#50075=CARTESIAN_POINT ( 'NONE',  ( 36.58470641641360999, -279.5969270664867281, -263.0529110095594092 ) ) ;
#50076=CARTESIAN_POINT ( 'NONE',  ( -92.43286910708727078, -283.2641184405466674, -219.3933482365070518 ) ) ;
#50077=CARTESIAN_POINT ( 'NONE',  ( -96.26953907633355811, -277.6893924657188109, -221.8617626637910689 ) ) ;
#50078=CARTESIAN_POINT ( 'NONE',  ( -30.89607534256120047, -285.0521122590863570, -193.9283342800665935 ) ) ;
#50079=CARTESIAN_POINT ( 'NONE',  ( -59.53433503689885953, -274.5602605802951643, -200.5937402867422463 ) ) ;
#50081=CARTESIAN_POINT ( 'NONE',  ( -84.35415942627538755, -292.9926427142486887, -213.4729022980585285 ) ) ;
#50082=CARTESIAN_POINT ( 'NONE',  ( 21.38625716607874949, -276.3148224881030615, -221.4772420431311275 ) ) ;
#50083=CARTESIAN_POINT ( 'NONE',  ( -40.51093074706013653, -276.7597824351230429, -343.3259228193078343 ) ) ;
#50084=CARTESIAN_POINT ( 'NONE',  ( -8.437181790818337745, -296.6739735600254448, -339.5815254536943826 ) ) ;
#50085=CARTESIAN_POINT ( 'NONE',  ( -74.68075533999848403, -291.7359748100731736, -203.0202317365652789 ) ) ;
#50086=CARTESIAN_POINT ( 'NONE',  ( 9.941316325251293051, -278.7771292210996990, -211.3565232439137560 ) ) ;
#50087=CARTESIAN_POINT ( 'NONE',  ( -19.38471394154651151, -292.1101746741380225, -195.4294187287191846 ) ) ;
#50088=CARTESIAN_POINT ( 'NONE',  ( -30.77397403837677103, -291.1959548843082075, -197.4209135535824942 ) ) ;
#50090=CARTESIAN_POINT ( 'NONE',  ( -67.44736475006726550, -293.4468762711809973, -339.0535455788008221 ) ) ;
#50093=CARTESIAN_POINT ( 'NONE',  ( -25.39285698143028114, -291.7160795765324792, -198.2317651843381441 ) ) ;
#50095=CARTESIAN_POINT ( 'NONE',  ( -53.28691492658257545, -277.3380690714490129, -200.3538533559491555 ) ) ;
#50096=CARTESIAN_POINT ( 'NONE',  ( -99.82399397337347580, -295.0173689200474882, -315.0464437874867940 ) ) ;
#50097=CARTESIAN_POINT ( 'NONE',  ( -76.49105543292736797, -284.8791118413384424, -336.1540047253961916 ) ) ;
#50098=CARTESIAN_POINT ( 'NONE',  ( 34.28374414271376480, -287.5723195959528198, -284.5252214534595510 ) ) ;
#50099=CARTESIAN_POINT ( 'NONE',  ( -9.710604166538601589, -278.2046676643375349, -338.6919445080791320 ) ) ;
#50100=CARTESIAN_POINT ( 'NONE',  ( 21.81156617014763555, -292.1991452502515472, -315.9093683592335537 ) ) ;
#50101=CARTESIAN_POINT ( 'NONE',  ( -45.17601688878938404, -296.9127319196196026, -344.0098322273660187 ) ) ;
#50102=CARTESIAN_POINT ( 'NONE',  ( 32.47115505635213140, -274.6460367698050504, -293.0171493173815520 ) ) ;
#50105=CARTESIAN_POINT ( 'NONE',  ( -107.7519723514942456, -296.6174498148145062, -239.1144293489067536 ) ) ;
#50106=CARTESIAN_POINT ( 'NONE',  ( -7.621527589300812089, -290.5798119572557425, -338.6659626074806511 ) ) ;
#50107=CARTESIAN_POINT ( 'NONE',  ( -75.31992539360024352, -295.5460990252308306, -205.6290498907350752 ) ) ;
#50108=CARTESIAN_POINT ( 'NONE',  ( -33.36826310765233217, -299.1804698133331613, -193.6695182843095608 ) ) ;
#50109=CARTESIAN_POINT ( 'NONE',  ( 35.55423826032691181, -288.2841963085366501, -276.4816238167906022 ) ) ;
#50111=CARTESIAN_POINT ( 'NONE',  ( -22.59958698792389242, -279.2950380960122061, -194.9711768236336979 ) ) ;
#50112=CARTESIAN_POINT ( 'NONE',  ( -56.03746276239288449, -295.9382499612493120, -344.9518764302059139 ) ) ;
#50113=CARTESIAN_POINT ( 'NONE',  ( -34.73345589466567418, -287.1592933305926181, -346.0810132864847333 ) ) ;
#50114=CARTESIAN_POINT ( 'NONE',  ( -93.67110267242016164, -296.1698454997695080, -322.8471171985851242 ) ) ;
#50115=CARTESIAN_POINT ( 'NONE',  ( 26.25088217052891437, -293.3930780179210274, -234.3681800691777539 ) ) ;
#50119=CARTESIAN_POINT ( 'NONE',  ( 9.370910816047025804, -288.2012664821090198, -210.0234039914137725 ) ) ;
#50120=CARTESIAN_POINT ( 'NONE',  ( -72.08107566293803359, -292.9809262143061233, -342.4248175857292154 ) ) ;
#50122=CARTESIAN_POINT ( 'NONE',  ( -39.57597471101205855, -279.3734097633271176, -193.4824822536768636 ) ) ;
#50123=CARTESIAN_POINT ( 'NONE',  ( -69.78142324358472592, -285.4804333033791295, -337.8118482579887427 ) ) ;
#50124=CARTESIAN_POINT ( 'NONE',  ( -73.31940589933238073, -284.1596851414851699, -202.8917585195025879 ) ) ;
#50125=CARTESIAN_POINT ( 'NONE',  ( -29.03626621203342850, -287.0259064076869890, -344.3363433242545284 ) ) ;
#50126=CARTESIAN_POINT ( 'NONE',  ( -14.93206348330923738, -278.6254446777232943, -342.7908673877399224 ) ) ;
#50127=CARTESIAN_POINT ( 'NONE',  ( -76.57916370595302169, -273.8443817128995761, -208.7777684575960961 ) ) ;
#50128=ORIENTED_EDGE ( 'NONE', *, *, #76364, .T. ) ;
#50129=CARTESIAN_POINT ( 'NONE',  ( -109.4920624883786360, -278.4056562853003243, -281.4663064671287884 ) ) ;
#50130=CARTESIAN_POINT ( 'NONE',  ( -69.77806339610459929, -278.9619490247505951, -204.8356139435566377 ) ) ;
#50131=CARTESIAN_POINT ( 'NONE',  ( -2.709484420801844706, -275.5788472459974514, -201.9205873271932887 ) ) ;
#50132=CARTESIAN_POINT ( 'NONE',  ( -71.04598935865531928, -278.4121359248661634, -201.5713686886269613 ) ) ;
#50133=CARTESIAN_POINT ( 'NONE',  ( 199.8333890556094445, 292.4321710294452146, -82.70894493957585780 ) ) ;
#50134=CARTESIAN_POINT ( 'NONE',  ( -68.75876545373007787, -274.5904350790960393, -200.3054333886574057 ) ) ;
#50136=CARTESIAN_POINT ( 'NONE',  ( -93.24416139441676421, -298.6936684336129133, -218.1924502067773517 ) ) ;
#50137=CARTESIAN_POINT ( 'NONE',  ( -114.2704648735229114, -281.0519495502701943, -270.3937649182068981 ) ) ;
#50141=CARTESIAN_POINT ( 'NONE',  ( -67.68815348001666621, -286.7239670075643403, -203.6279265148333479 ) ) ;
#50142=CARTESIAN_POINT ( 'NONE',  ( -109.9643034278956435, -286.5988573135857109, -247.8246976550084355 ) ) ;
#50143=CARTESIAN_POINT ( 'NONE',  ( 22.82909333039162192, -287.4783642228019858, -311.8966500789242104 ) ) ;
#50144=CARTESIAN_POINT ( 'NONE',  ( -113.0775286048948090, -283.8865432466141669, -284.2040875715013613 ) ) ;
#50145=CARTESIAN_POINT ( 'NONE',  ( 30.76755446176559872, -279.5749607082762509, -241.9433444497237531 ) ) ;
#50146=CARTESIAN_POINT ( 'NONE',  ( -52.36161242444706687, -287.7181875857285718, -197.6612712695019241 ) ) ;
#50147=CARTESIAN_POINT ( 'NONE',  ( 36.04468346152054181, -279.9371662121584450, -263.1021184434431461 ) ) ;
#50148=CARTESIAN_POINT ( 'NONE',  ( -4.832970197590103822, -277.9300333096678060, -336.2873630374841696 ) ) ;
#50149=CARTESIAN_POINT ( 'NONE',  ( 20.72662636625302568, -275.4212153638341078, -226.0002756500364569 ) ) ;
#50150=CARTESIAN_POINT ( 'NONE',  ( 9.970589359451627942, -287.2119452762335072, -330.6743853095651389 ) ) ;
#50152=CARTESIAN_POINT ( 'NONE',  ( -70.39137737591944699, -284.2795210547388933, -339.7432474565546272 ) ) ;
#50153=CARTESIAN_POINT ( 'NONE',  ( -83.84101961225024979, -284.1635088935872773, -331.7251853140549542 ) ) ;
#50154=CARTESIAN_POINT ( 'NONE',  ( 20.51462576511756808, -281.0920973096517059, -225.8251247738890868 ) ) ;
#50158=CARTESIAN_POINT ( 'NONE',  ( -62.33348748119884419, -291.2340923457712734, -341.9408250797640676 ) ) ;
#50159=CARTESIAN_POINT ( 'NONE',  ( -91.26292635598746017, -288.4839421182418846, -324.7108808063657079 ) ) ;
#50160=CARTESIAN_POINT ( 'NONE',  ( -40.77400899137278856, -273.0668063828048275, -197.1564365014620250 ) ) ;
#50162=CARTESIAN_POINT ( 'NONE',  ( 39.50471661373507715, -292.9360296936184795, -273.1790995700564508 ) ) ;
#50163=CARTESIAN_POINT ( 'NONE',  ( -102.2630339598794365, -288.5597252499873662, -305.3395242598816139 ) ) ;
#50164=CARTESIAN_POINT ( 'NONE',  ( 24.19606324295878963, -291.2287696727721595, -229.2384029351687786 ) ) ;
#50165=CARTESIAN_POINT ( 'NONE',  ( 20.64497273588014536, -288.1268572152636693, -225.3647150568420159 ) ) ;
#50166=CARTESIAN_POINT ( 'NONE',  ( -110.4542110544635705, -286.8376638359844719, -287.0812184334320705 ) ) ;
#50167=CARTESIAN_POINT ( 'NONE',  ( 29.90575366690926984, -289.9917707621133331, -303.6864665132742971 ) ) ;
#50168=CARTESIAN_POINT ( 'NONE',  ( -110.7797619687470956, -288.3466611540799249, -286.3885789207768084 ) ) ;
#50169=CARTESIAN_POINT ( 'NONE',  ( -35.89714563425030747, -294.0703967668365522, -195.3623998638208548 ) ) ;
#50170=CARTESIAN_POINT ( 'NONE',  ( -65.39477605066088017, -284.3693414041481446, -338.0241005783956325 ) ) ;
#50171=CARTESIAN_POINT ( 'NONE',  ( 24.95875597068581087, -294.9835569251786751, -228.2139041085275153 ) ) ;
#50175=CARTESIAN_POINT ( 'NONE',  ( -105.3694235135199904, -274.9566242683296196, -237.9476076708264429 ) ) ;
#50176=CARTESIAN_POINT ( 'NONE',  ( -36.20124657383839661, -282.2346565089146679, -343.5137057234255735 ) ) ;
#50177=CARTESIAN_POINT ( 'NONE',  ( -90.32473010579826678, -281.8011817670309256, -323.5169858690355227 ) ) ;
#50178=CARTESIAN_POINT ( 'NONE',  ( -68.17079532744206460, -294.6440106118486142, -340.7438268683401930 ) ) ;
#50179=CARTESIAN_POINT ( 'NONE',  ( 23.90328057740336831, -273.2217536208866591, -228.7808688120199463 ) ) ;
#50180=CARTESIAN_POINT ( 'NONE',  ( -92.04230275899415403, -275.9202631479766978, -320.9253149356404720 ) ) ;
#50181=CARTESIAN_POINT ( 'NONE',  ( -69.48826278308541760, -298.9350781951204681, -204.2714668322632576 ) ) ;
#50182=CARTESIAN_POINT ( 'NONE',  ( 10.68972029633187937, -295.7980480551170785, -326.1137642656909179 ) ) ;
#50184=CARTESIAN_POINT ( 'NONE',  ( -42.39068516581224344, -295.9202903350091560, -343.3481680476940028 ) ) ;
#50186=CARTESIAN_POINT ( 'NONE',  ( 38.05633600158335383, -285.5874632921277794, -271.5510281369199106 ) ) ;
#50187=CARTESIAN_POINT ( 'NONE',  ( -105.8058295604936063, -296.8916587374533265, -244.8842449792233822 ) ) ;
#50188=CARTESIAN_POINT ( 'NONE',  ( 38.95487779611155332, -287.0909434536848153, -260.1348533389456179 ) ) ;
#50189=CARTESIAN_POINT ( 'NONE',  ( 21.02892139838816021, -296.1858743455904914, -318.0393037442775039 ) ) ;
#50190=CARTESIAN_POINT ( 'NONE',  ( 37.02594314257099484, -291.6650951413106441, -279.1505413507780418 ) ) ;
#50191=CARTESIAN_POINT ( 'NONE',  ( -61.98614075014549485, -278.9370407720724074, -197.5258170954137711 ) ) ;
#50192=CARTESIAN_POINT ( 'NONE',  ( -20.25526795762938548, -286.3380690714490697, -345.3683826091709648 ) ) ;
#50193=CARTESIAN_POINT ( 'NONE',  ( 17.19589066053204007, -285.6473943493583647, -221.2222758851342235 ) ) ;
#50196=CARTESIAN_POINT ( 'NONE',  ( -109.8353168242309010, -298.3335539051417982, -256.4692476335356446 ) ) ;
#50197=CARTESIAN_POINT ( 'NONE',  ( -17.16518032620580669, -281.7329341780680920, -196.6623097148463160 ) ) ;
#50198=CARTESIAN_POINT ( 'NONE',  ( -112.6929954034260390, -294.5820657255896435, -269.5935894327433857 ) ) ;
#50199=CARTESIAN_POINT ( 'NONE',  ( 35.70282396646855716, -281.5647190748069306, -271.3137581944124008 ) ) ;
#50200=CARTESIAN_POINT ( 'NONE',  ( -114.2336749270550769, -296.6565454245620117, -275.3414882687744125 ) ) ;
#50201=CARTESIAN_POINT ( 'NONE',  ( -107.7656868571581157, -274.2599289040125541, -248.8360794169643100 ) ) ;
#50202=CARTESIAN_POINT ( 'NONE',  ( -35.16475450806476033, -284.1591034817870423, -194.8195829246140534 ) ) ;
#50203=CARTESIAN_POINT ( 'NONE',  ( 34.25858975496183234, -283.2643670651485195, -248.0362632730956136 ) ) ;
#50204=CARTESIAN_POINT ( 'NONE',  ( -94.62790106707559801, -296.2531683619527030, -224.7354713465992120 ) ) ;
#50208=CARTESIAN_POINT ( 'NONE',  ( -54.03348678089458446, -285.2472652557833044, -343.1689661315664921 ) ) ;
#50210=CARTESIAN_POINT ( 'NONE',  ( 31.95455697924147032, -291.4809262143061233, -303.7686719486574702 ) ) ;
#50211=CARTESIAN_POINT ( 'NONE',  ( 27.50704705598299782, -275.2917780826409171, -311.6764883431170574 ) ) ;
#50212=CARTESIAN_POINT ( 'NONE',  ( -44.29809233384927580, -291.7951796514071816, -197.6425038824307876 ) ) ;
#50214=CARTESIAN_POINT ( 'NONE',  ( 0.7418328627382330120, -282.0897158423945825, -207.2120225293148508 ) ) ;
#50215=CARTESIAN_POINT ( 'NONE',  ( -4.694036087942145663, -278.2149415568750896, -336.5610401846183777 ) ) ;
#50216=CARTESIAN_POINT ( 'NONE',  ( 27.63362223826922559, -283.6789670515210560, -310.2687905128263424 ) ) ;
#50217=CARTESIAN_POINT ( 'NONE',  ( 18.27539814306031829, -279.6684910955020200, -222.4474687750023350 ) ) ;
#50218=CARTESIAN_POINT ( 'NONE',  ( -110.2394639135455208, -280.7787490049236112, -252.7282881482385619 ) ) ;
#50219=CARTESIAN_POINT ( 'NONE',  ( -20.50992399667585886, -298.2574375460679335, -193.3611160711894854 ) ) ;
#50220=CARTESIAN_POINT ( 'NONE',  ( 20.81885638852990184, -276.0675619174349436, -320.8424411334291335 ) ) ;
#50221=CARTESIAN_POINT ( 'NONE',  ( 20.83417430341074095, -296.1158046415303602, -316.8236891720168273 ) ) ;
#50224=CARTESIAN_POINT ( 'NONE',  ( 3.540531325833613074, -292.6486151179939839, -334.2111870952561503 ) ) ;
#50225=CARTESIAN_POINT ( 'NONE',  ( 20.73426050244066587, -274.4366802819465647, -226.0102708529038296 ) ) ;
#50226=CARTESIAN_POINT ( 'NONE',  ( 37.37900150782583353, -294.8761462264361626, -254.8205746371423004 ) ) ;
#50227=CARTESIAN_POINT ( 'NONE',  ( -8.674131915659689440, -293.6241456497128297, -199.3246537432844718 ) ) ;
#50228=CARTESIAN_POINT ( 'NONE',  ( -70.76904965004152359, -291.4942087341351566, -337.3278481484095437 ) ) ;
#50229=CARTESIAN_POINT ( 'NONE',  ( -110.8488235094794163, -276.3706251407230639, -284.4550345326309184 ) ) ;
#50230=CARTESIAN_POINT ( 'NONE',  ( -10.71659673397097734, -278.6223347687520686, -339.8767138388106446 ) ) ;
#50232=CARTESIAN_POINT ( 'NONE',  ( -26.01189438197866366, -292.9866028714436652, -343.9338690352085450 ) ) ;
#50233=CARTESIAN_POINT ( 'NONE',  ( 28.69708180864721214, -283.9034567176025234, -307.6054775750404815 ) ) ;
#50234=CARTESIAN_POINT ( 'NONE',  ( -70.10830499006489447, -284.5303195975483845, -204.7683412375857301 ) ) ;
#50236=CARTESIAN_POINT ( 'NONE',  ( -2.422284508983608031, -282.2433995548834673, -334.5059178052410971 ) ) ;
#50237=CARTESIAN_POINT ( 'NONE',  ( -73.63155621386408711, -280.6617505313870993, -202.7848550276897868 ) ) ;
#50238=CARTESIAN_POINT ( 'NONE',  ( -80.70074920807873298, -284.2735415023436190, -207.1464733336419783 ) ) ;
#50239=CARTESIAN_POINT ( 'NONE',  ( -109.3895241792176733, -279.8310018279798896, -243.7136017212736476 ) ) ;
#50240=CARTESIAN_POINT ( 'NONE',  ( -68.71248336467130002, -278.9771483566601091, -339.9353054930013514 ) ) ;
#50241=CARTESIAN_POINT ( 'NONE',  ( 17.36665895637874613, -295.4090924074130839, -226.6919474004047572 ) ) ;
#50244=CARTESIAN_POINT ( 'NONE',  ( -83.18623497663864441, -299.4249573779193270, -210.9380631999358968 ) ) ;
#50245=CARTESIAN_POINT ( 'NONE',  ( -36.97551065040104845, -278.0768702752188801, -195.7172119192860862 ) ) ;
#50246=CARTESIAN_POINT ( 'NONE',  ( -50.41435204032848816, -293.6475800832835148, -195.5073954061652444 ) ) ;
#50247=CARTESIAN_POINT ( 'NONE',  ( 25.87666342129961805, -293.4036242026455739, -307.0671280911795407 ) ) ;
#50248=CARTESIAN_POINT ( 'NONE',  ( -113.9449388050913825, -290.1564855603656952, -262.6368981308480670 ) ) ;
#50250=CARTESIAN_POINT ( 'NONE',  ( 37.48983357727624366, -292.3216586563302144, -285.8158214122535696 ) ) ;
#50251=CARTESIAN_POINT ( 'NONE',  ( -30.43635620055726676, -284.5406554786366655, -196.8335303357073087 ) ) ;
#50252=CARTESIAN_POINT ( 'NONE',  ( -88.80365871201126993, -293.1810922391674126, -216.7874161164737643 ) ) ;
#50253=CARTESIAN_POINT ( 'NONE',  ( -42.95397476381405966, -284.4395045866243095, -343.6900928545240959 ) ) ;
#50254=CARTESIAN_POINT ( 'NONE',  ( -111.3120250584146191, -291.2354814739172753, -290.8845495444705875 ) ) ;
#50255=CARTESIAN_POINT ( 'NONE',  ( -30.26265832149410073, -280.6363286675345989, -197.5929399114839669 ) ) ;
#50256=CARTESIAN_POINT ( 'NONE',  ( 39.04626408082600619, -292.2749854261301721, -264.6263432063596497 ) ) ;
#50257=CARTESIAN_POINT ( 'NONE',  ( -70.55998728160321321, -290.2818027360690962, -339.6626870678834393 ) ) ;
#50258=CARTESIAN_POINT ( 'NONE',  ( -111.8608620435123697, -290.8041557688309240, -289.5559425867264167 ) ) ;
#50259=CARTESIAN_POINT ( 'NONE',  ( -106.5329923461504791, -285.0298482026460078, -246.9312712180887104 ) ) ;
#50262=CARTESIAN_POINT ( 'NONE',  ( 38.20757594392513568, -295.3399833929092893, -264.6503944321192989 ) ) ;
#50263=CARTESIAN_POINT ( 'NONE',  ( -97.89448193200388459, -294.6088082618283579, -317.1228426132867639 ) ) ;
#50264=CARTESIAN_POINT ( 'NONE',  ( -91.46264729407023708, -278.3161502095563833, -221.0221726530852777 ) ) ;
#50266=CARTESIAN_POINT ( 'NONE',  ( -95.97671714198153836, -272.7320661652116200, -220.5265633770405032 ) ) ;
#50267=CARTESIAN_POINT ( 'NONE',  ( -95.33090054539448488, -294.3968480552210281, -315.8359504680674945 ) ) ;
#50268=CARTESIAN_POINT ( 'NONE',  ( 32.06085759139318725, -276.9740805369317513, -244.6461613591418995 ) ) ;
#50269=CARTESIAN_POINT ( 'NONE',  ( -83.94798291180906347, -271.5435275721050061, -212.5794610098595285 ) ) ;
#50271=CARTESIAN_POINT ( 'NONE',  ( 34.60267695094090357, -294.5665856550675699, -255.8305600918416758 ) ) ;
#50272=CARTESIAN_POINT ( 'NONE',  ( -95.84273018092272878, -297.0135626204751702, -314.5616018979806654 ) ) ;
#50275=CARTESIAN_POINT ( 'NONE',  ( -111.5748610248523249, -294.7043319690050112, -258.4701674731024355 ) ) ;
#50276=CARTESIAN_POINT ( 'NONE',  ( -75.73621665072249698, -298.2054887986585641, -203.6728771563084592 ) ) ;
#50277=CARTESIAN_POINT ( 'NONE',  ( 33.64550499664232319, -286.3832993171898806, -289.9456977756863125 ) ) ;
#50278=CARTESIAN_POINT ( 'NONE',  ( -60.10630012970916169, -275.7573956496621577, -198.8450460799258224 ) ) ;
#50279=CARTESIAN_POINT ( 'NONE',  ( -110.6034901111379440, -291.5183084014535666, -268.4675968260048080 ) ) ;
#50280=CARTESIAN_POINT ( 'NONE',  ( -73.92113913693324889, -274.0723617322286145, -202.6153224273677722 ) ) ;
#50282=CARTESIAN_POINT ( 'NONE',  ( -99.91710299353974278, -297.4042943384935143, -232.6276017677705568 ) ) ;
#50284=CARTESIAN_POINT ( 'NONE',  ( -109.8508240012940149, -280.2693194364147189, -290.8753510809888212 ) ) ;
#50285=CARTESIAN_POINT ( 'NONE',  ( 35.70984346184874170, -279.9495675700271136, -247.6285366970083714 ) ) ;
#50287=CARTESIAN_POINT ( 'NONE',  ( -16.17786546318904684, -282.1342298324216813, -344.3447053673556297 ) ) ;
#50288=CARTESIAN_POINT ( 'NONE',  ( 39.27823336103507046, -274.9825707383294571, -276.8955329131857184 ) ) ;
#50289=CARTESIAN_POINT ( 'NONE',  ( -92.48064189481800668, -277.6793742011579980, -217.6916684475944805 ) ) ;
#50290=CARTESIAN_POINT ( 'NONE',  ( -58.75490761657733430, -277.7756543150019866, -198.3090328693548940 ) ) ;
#50292=CARTESIAN_POINT ( 'NONE',  ( -75.45214434226805622, -296.2175574461771816, -207.4623457955987362 ) ) ;
#50293=CARTESIAN_POINT ( 'NONE',  ( 22.97339870047947130, -278.1607918486978406, -314.9591988313621869 ) ) ;
#50295=CARTESIAN_POINT ( 'NONE',  ( -61.14460228282200660, -289.7648841358002301, -198.8091138861177569 ) ) ;
#50296=CARTESIAN_POINT ( 'NONE',  ( -100.0310483308176828, -291.1443451806417784, -225.6504299771615365 ) ) ;
#50297=CARTESIAN_POINT ( 'NONE',  ( -16.31521333151226827, -276.3233417229643578, -198.1412156074836446 ) ) ;
#50298=CARTESIAN_POINT ( 'NONE',  ( -110.4797419884152845, -270.7652409156175395, -253.7530631127523577 ) ) ;
#50299=CARTESIAN_POINT ( 'NONE',  ( -107.7740140549030770, -284.1432294191976098, -239.5125219399257901 ) ) ;
#50301=CARTESIAN_POINT ( 'NONE',  ( -110.5914043820631605, -282.3444769689195937, -286.5279133427056308 ) ) ;
#50304=CARTESIAN_POINT ( 'NONE',  ( 22.13543961663703996, -291.7484484370533551, -227.3327597997061105 ) ) ;
#50305=CARTESIAN_POINT ( 'NONE',  ( -38.62285886196762164, -284.1755375516056006, -196.1242769990700197 ) ) ;
#50308=CARTESIAN_POINT ( 'NONE',  ( -56.33370758817049051, -293.2965588918303297, -342.9704675057781742 ) ) ;
#50309=CARTESIAN_POINT ( 'NONE',  ( -111.5494764710839917, -282.8070314947411248, -288.1904484659032164 ) ) ;
#50310=CARTESIAN_POINT ( 'NONE',  ( -97.06497439797817606, -280.7524148827258728, -227.0070994037915568 ) ) ;
#50311=CARTESIAN_POINT ( 'NONE',  ( -113.4270414053005425, -285.8689813377288260, -261.4712607929455999 ) ) ;
#50312=CARTESIAN_POINT ( 'NONE',  ( -9.215084572556941467, -278.6547507738487184, -199.7716888058341453 ) ) ;
#50313=CARTESIAN_POINT ( 'NONE',  ( 26.36738027536458873, -287.0634180033556504, -234.6184865306303209 ) ) ;
#50314=CARTESIAN_POINT ( 'NONE',  ( -110.4876238152767485, -279.8660062091835243, -278.8758744569841497 ) ) ;
#50315=CARTESIAN_POINT ( 'NONE',  ( -109.4434800205092984, -279.1907055100448929, -282.8421648300742959 ) ) ;
#50316=CARTESIAN_POINT ( 'NONE',  ( -10.60172030037941404, -288.3789836559200808, -199.8542767404049982 ) ) ;
#50318=CARTESIAN_POINT ( 'NONE',  ( -26.20759799648282851, -298.0212679064690633, -193.3614219870460147 ) ) ;
#50319=CARTESIAN_POINT ( 'NONE',  ( -7.539123811414215837, -290.6395404315176165, -338.8536064857112819 ) ) ;
#50321=CARTESIAN_POINT ( 'NONE',  ( -99.86837403722181250, -286.4090924074130839, -320.2651865833026363 ) ) ;
#50323=CARTESIAN_POINT ( 'NONE',  ( -54.88053346861718040, -271.8270095330213962, -197.2692733724240384 ) ) ;
#50324=CARTESIAN_POINT ( 'NONE',  ( 35.94046486524361228, -291.6869468967016701, -249.4289712438227298 ) ) ;
#50325=CARTESIAN_POINT ( 'NONE',  ( 36.34866108994013700, -289.0809342277619294, -271.0232464093949716 ) ) ;
#50326=CARTESIAN_POINT ( 'NONE',  ( 35.05171798619566914, -283.1111659630980171, -254.9005914110520905 ) ) ;
#50327=CARTESIAN_POINT ( 'NONE',  ( 9.878179787375804821, -289.8418700464339395, -330.5024744715683482 ) ) ;
#50328=CARTESIAN_POINT ( 'NONE',  ( 36.67161757024006619, -289.1113873841904933, -289.7344779729380093 ) ) ;
#50329=CARTESIAN_POINT ( 'NONE',  ( -109.6837122555746191, -286.2972642358467397, -290.1992865056311075 ) ) ;
#50330=CARTESIAN_POINT ( 'NONE',  ( -113.7659728382104447, -278.5960129198955997, -280.1816053145672072 ) ) ;
#50332=CARTESIAN_POINT ( 'NONE',  ( -50.24610959810592448, -293.2953341788693820, -344.8639751174833918 ) ) ;
#50333=CARTESIAN_POINT ( 'NONE',  ( 39.52902354657486939, -281.4517800365271682, -275.6630135752549791 ) ) ;
#50335=CARTESIAN_POINT ( 'NONE',  ( 97.65637974683852462, -301.6750618930004748, -195.8765629805787682 ) ) ;
#50336=CARTESIAN_POINT ( 'NONE',  ( 10.64812456238590066, -284.9090924074130271, -330.4860931364851808 ) ) ;
#50337=CARTESIAN_POINT ( 'NONE',  ( -92.42198639639629221, -271.5171745323133905, -217.9958269592325166 ) ) ;
#50340=CARTESIAN_POINT ( 'NONE',  ( -72.15351379383706387, -279.0860899361107954, -206.1261892359662511 ) ) ;
#50342=CARTESIAN_POINT ( 'NONE',  ( -14.69237671000794521, -277.9702099961260160, -343.5946400563753969 ) ) ;
#50343=CARTESIAN_POINT ( 'NONE',  ( -35.14369412956378369, -299.5054696142980220, -196.7713390149831696 ) ) ;
#50344=CARTESIAN_POINT ( 'NONE',  ( -112.9075215949943782, -283.4377109778860131, -284.1671756000792470 ) ) ;
#50345=CARTESIAN_POINT ( 'NONE',  ( -103.3229610897474373, -292.7628101456688228, -236.7148213140268069 ) ) ;
#50346=CARTESIAN_POINT ( 'NONE',  ( -52.40759924451852925, -275.4625770938109213, -195.6114626430798182 ) ) ;
#50348=CARTESIAN_POINT ( 'NONE',  ( -64.73922498883916887, -275.0169447323681311, -198.9140188814967019 ) ) ;
#50349=CARTESIAN_POINT ( 'NONE',  ( 37.36314606568671337, -295.4854416488993252, -265.1642700852298162 ) ) ;
#50350=CARTESIAN_POINT ( 'NONE',  ( -93.04636888076693424, -281.8542081291388968, -320.3505817338285624 ) ) ;
#50352=CARTESIAN_POINT ( 'NONE',  ( -90.76820565737011748, -290.9863102207815473, -214.8673551589249371 ) ) ;
#50353=CARTESIAN_POINT ( 'NONE',  ( -16.15009226224445626, -272.3474548112154139, -198.7337390904931738 ) ) ;
#50354=CARTESIAN_POINT ( 'NONE',  ( -49.24012302223133730, -287.5032021760997623, -195.0426219151532052 ) ) ;
#50355=CARTESIAN_POINT ( 'NONE',  ( -110.0046263325880034, -289.6049936938659357, -260.2730099703517794 ) ) ;
#50357=CARTESIAN_POINT ( 'NONE',  ( -91.19622158036550275, -288.3738615785473485, -324.6416262466795501 ) ) ;
#50358=CARTESIAN_POINT ( 'NONE',  ( -39.96306329981003103, -288.7525814210067097, -343.3847879840174642 ) ) ;
#50360=CARTESIAN_POINT ( 'NONE',  ( -18.27223636199831702, -287.3718466160934213, -196.0240202023492202 ) ) ;
#50362=CARTESIAN_POINT ( 'NONE',  ( -27.01432979943238522, -277.2505004070605992, -342.6482738873991707 ) ) ;
#50364=CARTESIAN_POINT ( 'NONE',  ( 30.63134982468524470, -292.0111811076992581, -234.7339838467658240 ) ) ;
#50365=CARTESIAN_POINT ( 'NONE',  ( -114.2388749865937285, -285.2082041814914533, -269.9905980131128445 ) ) ;
#50366=CARTESIAN_POINT ( 'NONE',  ( -111.4699639621629217, -284.6252924125633399, -291.1155101083857062 ) ) ;
#50367=CARTESIAN_POINT ( 'NONE',  ( -51.83570800445956195, -280.1949714541942171, -198.7411442248631772 ) ) ;
#50368=CARTESIAN_POINT ( 'NONE',  ( 154.3179510270316825, 206.9283153158852997, -217.4371041850278630 ) ) ;
#50369=CARTESIAN_POINT ( 'NONE',  ( -72.06973415904727176, -195.5151140978756246, -359.6196184014357300 ) ) ;
#50370=CARTESIAN_POINT ( 'NONE',  ( -109.3056031691116488, -263.8853751231396814, -305.5667918931541749 ) ) ;
#50371=CARTESIAN_POINT ( 'NONE',  ( -14.00427616992897839, -273.5599878219673542, -201.0216171930390772 ) ) ;
#50372=CARTESIAN_POINT ( 'NONE',  ( 34.42677511111907052, -274.2752844536925636, -255.3494618599178523 ) ) ;
#50373=CARTESIAN_POINT ( 'NONE',  ( -105.9057119658662884, -295.6086158138003270, -305.3855614695280565 ) ) ;
#50374=CARTESIAN_POINT ( 'NONE',  ( -109.1997399844073584, -269.5207596422944789, -295.4475377585682736 ) ) ;
#50375=CARTESIAN_POINT ( 'NONE',  ( -43.98314901247594833, -272.6548208346287652, -194.0901128034429064 ) ) ;
#50376=CARTESIAN_POINT ( 'NONE',  ( -72.26672099815004913, -299.4454364413379608, -204.8401254970598870 ) ) ;
#50377=CARTESIAN_POINT ( 'NONE',  ( 34.18488191215580940, -289.0886210737508577, -287.2487330086863153 ) ) ;
#50379=CARTESIAN_POINT ( 'NONE',  ( -113.9980744054674631, -297.4309926713159484, -275.3361058418064999 ) ) ;
#50380=CARTESIAN_POINT ( 'NONE',  ( -70.01557291589455190, -286.1020837837185127, -204.9988144284792497 ) ) ;
#50381=CARTESIAN_POINT ( 'NONE',  ( -67.40176349790807819, -272.5873438394476125, -199.8069891131355291 ) ) ;
#50383=CARTESIAN_POINT ( 'NONE',  ( 36.92387453727684488, -294.1070301515349570, -250.5927937790800684 ) ) ;
#50384=CARTESIAN_POINT ( 'NONE',  ( 6.584014889699429496, -294.9652480824167924, -333.5929473193716035 ) ) ;
#50385=CARTESIAN_POINT ( 'NONE',  ( -79.53243520000641809, -291.6313249584576965, -210.7261612519274649 ) ) ;
#50386=ORIENTED_EDGE ( 'NONE', *, *, #28465, .F. ) ;
#50387=CARTESIAN_POINT ( 'NONE',  ( -75.72275237452288366, -275.4646790912669871, -205.2144843793558948 ) ) ;
#50390=CARTESIAN_POINT ( 'NONE',  ( -112.1168617958987568, -277.8323660846900225, -288.5326667410064942 ) ) ;
#50391=CARTESIAN_POINT ( 'NONE',  ( 35.49336973230709447, -274.1112568995672518, -282.5644690008441557 ) ) ;
#50392=CARTESIAN_POINT ( 'NONE',  ( -37.84053400009924673, -299.2508443843946111, -196.9657388980841404 ) ) ;
#50393=CARTESIAN_POINT ( 'NONE',  ( 33.12752987348345357, -276.7566769568019822, -290.3443410881425280 ) ) ;
#50394=CARTESIAN_POINT ( 'NONE',  ( 36.64306673344027132, -277.0920454183344646, -252.9774930820295538 ) ) ;
#50395=CARTESIAN_POINT ( 'NONE',  ( -26.04203593737108591, -274.9290531893300340, -344.8643017382003109 ) ) ;
#50396=CARTESIAN_POINT ( 'NONE',  ( -15.55454980169585788, -295.4141749147962059, -340.1941099898121479 ) ) ;
#50397=CARTESIAN_POINT ( 'NONE',  ( -4.086493197662068866, -293.1795092828187421, -336.0217518665535295 ) ) ;
#50399=CARTESIAN_POINT ( 'NONE',  ( -113.6568941996796269, -279.1719006691246250, -260.1822273235796388 ) ) ;
#50400=CARTESIAN_POINT ( 'NONE',  ( -36.46404459810915455, -277.2075663479450327, -343.3683091744609328 ) ) ;
#50401=CARTESIAN_POINT ( 'NONE',  ( -3.691058235656173192, -285.1717261881592549, -201.6376383291749335 ) ) ;
#50402=CARTESIAN_POINT ( 'NONE',  ( -100.7830366863755955, -299.0935691332473425, -230.0470355627635115 ) ) ;
#50403=CARTESIAN_POINT ( 'NONE',  ( 82.62320746513702829, -301.5722161194245245, -196.8457140964393943 ) ) ;
#50405=CARTESIAN_POINT ( 'NONE',  ( 22.08690161819221842, -287.3445316385027581, -313.0324552212792355 ) ) ;
#50407=CARTESIAN_POINT ( 'NONE',  ( -79.22363092633919734, -275.8653573966271892, -331.4471224264939337 ) ) ;
#50408=CARTESIAN_POINT ( 'NONE',  ( -78.98023517226346257, -276.2001724052498730, -331.0994277800444365 ) ) ;
#50409=CARTESIAN_POINT ( 'NONE',  ( -20.07103143784055632, -284.8305155240813065, -343.3982667085224989 ) ) ;
#50410=CARTESIAN_POINT ( 'NONE',  ( -48.65397875235746739, -278.4043432548106125, -342.9328708925188494 ) ) ;
#50413=CARTESIAN_POINT ( 'NONE',  ( 30.54688990539132476, -273.5016753868712840, -235.7550526658807541 ) ) ;
#50415=CARTESIAN_POINT ( 'NONE',  ( 25.35899675022165667, -275.6861437755006818, -232.6796445339590775 ) ) ;
#50416=CARTESIAN_POINT ( 'NONE',  ( 29.45978265135702401, -284.0073380408512094, -304.8225503676121662 ) ) ;
#50418=CARTESIAN_POINT ( 'NONE',  ( 0.02878841654864764885, -290.4793893536851783, -336.0918662167628099 ) ) ;
#50420=CARTESIAN_POINT ( 'NONE',  ( 29.79767475420488054, -291.1094346075341832, -236.8199325610007691 ) ) ;
#50422=CARTESIAN_POINT ( 'NONE',  ( -110.8348508120440101, -271.2371897950222888, -270.3444116073703185 ) ) ;
#50423=CARTESIAN_POINT ( 'NONE',  ( -4.261730838314683467, -290.6324690631940371, -203.8895927681387548 ) ) ;
#50424=CARTESIAN_POINT ( 'NONE',  ( -108.4555765497910471, -262.4588243622614527, -317.8183916042563055 ) ) ;
#50426=CARTESIAN_POINT ( 'NONE',  ( -62.55301335731594747, -287.8540992579118551, -342.4385068502485296 ) ) ;
#50427=CARTESIAN_POINT ( 'NONE',  ( -68.09941197489402498, -285.0630646150916050, -337.4461653420434004 ) ) ;
#50428=CARTESIAN_POINT ( 'NONE',  ( -87.06963639359018714, -283.6109735456283829, -212.8362216305413597 ) ) ;
#50429=CIRCLE ( 'NONE', #21715, 6.154241149514405151 ) ;
#50430=CARTESIAN_POINT ( 'NONE',  ( -91.16010416744582301, -285.2614126684633220, -320.5503031129671854 ) ) ;
#50432=CARTESIAN_POINT ( 'NONE',  ( -110.0319674729293808, -285.2401243299765952, -279.0877432656427573 ) ) ;
#50433=CARTESIAN_POINT ( 'NONE',  ( -61.19241030814799132, -293.7240306000317673, -198.8250346200564138 ) ) ;
#50434=CARTESIAN_POINT ( 'NONE',  ( -64.89647830068022927, -274.0352103075979358, -198.4687159848319027 ) ) ;
#50436=CARTESIAN_POINT ( 'NONE',  ( -81.07662245399937717, -289.5429708344407800, -208.7447990020838233 ) ) ;
#50437=CARTESIAN_POINT ( 'NONE',  ( -56.92402925571688144, -277.2978082133980138, -344.8845020303465390 ) ) ;
#50438=CARTESIAN_POINT ( 'NONE',  ( 36.84450477800405821, -295.6445062859062318, -279.0781348419051255 ) ) ;
#50440=CARTESIAN_POINT ( 'NONE',  ( -85.33152481854864391, -293.9090924074130839, -210.2361428286349110 ) ) ;
#50441=CARTESIAN_POINT ( 'NONE',  ( -110.8017595996040257, -283.2658667256583271, -268.1558653716044205 ) ) ;
#50442=CARTESIAN_POINT ( 'NONE',  ( -81.05204825041448657, -277.4582436470126936, -209.4151902017766815 ) ) ;
#50443=CARTESIAN_POINT ( 'NONE',  ( -43.96312658206134216, -272.4499059399690850, -194.2894473756018670 ) ) ;
#50444=CARTESIAN_POINT ( 'NONE',  ( 32.16131357893130627, -274.5986080161726477, -247.5437793123001882 ) ) ;
#50445=CARTESIAN_POINT ( 'NONE',  ( -17.26210013418049272, -293.8360477393512156, -199.4030420448374628 ) ) ;
#50446=VECTOR ( 'NONE', #56887, 999.9999999999998863 ) ;
#50447=CARTESIAN_POINT ( 'NONE',  ( -7.184270956131327601, -293.3990244232187479, -203.6232882716992663 ) ) ;
#50448=CARTESIAN_POINT ( 'NONE',  ( 30.47301169727677816, -295.3272022080167858, -305.7795190125078761 ) ) ;
#50449=CARTESIAN_POINT ( 'NONE',  ( -103.9374875671850020, -295.9812336854413388, -300.3845429058175682 ) ) ;
#50450=CARTESIAN_POINT ( 'NONE',  ( -76.90265548686402042, -291.5822160142303119, -334.0787094229563081 ) ) ;
#50451=CARTESIAN_POINT ( 'NONE',  ( -74.27411833339516534, -283.6955025699494968, -337.9853668908753548 ) ) ;
#50452=CARTESIAN_POINT ( 'NONE',  ( -4.342332206735987299, -272.6220107447962846, -202.1460536848136940 ) ) ;
#50453=CARTESIAN_POINT ( 'NONE',  ( 37.72010669771049152, -287.1701095952975606, -253.1350320327633199 ) ) ;
#50454=CARTESIAN_POINT ( 'NONE',  ( -101.9951472667570300, -280.0305432084947483, -307.7714173920122676 ) ) ;
#50455=CARTESIAN_POINT ( 'NONE',  ( -49.44866146962257147, -284.9528909403255739, -198.0818289740959131 ) ) ;
#50456=CARTESIAN_POINT ( 'NONE',  ( -105.9134105031455135, -288.1525095434603827, -300.8685683642787581 ) ) ;
#50457=CARTESIAN_POINT ( 'NONE',  ( 192.1331913634949160, 286.0196433216794389, -110.9393339982713940 ) ) ;
#50458=CARTESIAN_POINT ( 'NONE',  ( -106.5886274555256392, -284.3709272072370027, -246.9035698887442720 ) ) ;
#50459=CARTESIAN_POINT ( 'NONE',  ( 37.59302098626444888, -282.5565572778405112, -254.3988544766780819 ) ) ;
#50460=CARTESIAN_POINT ( 'NONE',  ( -98.84782537177314055, -288.9977118160620648, -316.3156013001191695 ) ) ;
#50461=CARTESIAN_POINT ( 'NONE',  ( -111.6992376003494201, -279.9417900779183128, -287.0163585937223161 ) ) ;
#50462=CARTESIAN_POINT ( 'NONE',  ( -112.5147846417367674, -280.0472341064390776, -256.0675557195702368 ) ) ;
#50463=CARTESIAN_POINT ( 'NONE',  ( -14.30686415809234902, -280.1925111863634470, -201.0372202223673241 ) ) ;
#50464=CARTESIAN_POINT ( 'NONE',  ( -75.12727705376188680, -275.5263574673310245, -205.9265705689643369 ) ) ;
#50465=CARTESIAN_POINT ( 'NONE',  ( 19.41566216221196584, -292.8442308958108811, -218.3264965671178572 ) ) ;
#50466=CARTESIAN_POINT ( 'NONE',  ( 25.61230844166575338, -286.1146300050408513, -310.4689676739845936 ) ) ;
#50467=CARTESIAN_POINT ( 'NONE',  ( -69.30635844397487233, -293.2387339056230076, -201.1753907227580100 ) ) ;
#50468=CARTESIAN_POINT ( 'NONE',  ( -106.0909435701332484, -295.8121612422846738, -244.7634910073658716 ) ) ;
#50469=CARTESIAN_POINT ( 'NONE',  ( 21.33077079710802693, -284.1055228959285728, -316.1743841523888818 ) ) ;
#50470=CARTESIAN_POINT ( 'NONE',  ( -70.94430627564580050, -295.1750121629748946, -335.2052875502798202 ) ) ;
#50471=CARTESIAN_POINT ( 'NONE',  ( -0.9626585369666372793, -293.6032557839350261, -202.8477278792764764 ) ) ;
#50472=CARTESIAN_POINT ( 'NONE',  ( 35.53135705636167074, -282.2877554778768854, -276.7518076517758345 ) ) ;
#50474=CARTESIAN_POINT ( 'NONE',  ( 7.776902166684397599, -297.5249256984344584, -193.6782679355795267 ) ) ;
#50475=CARTESIAN_POINT ( 'NONE',  ( -37.49305186129453915, -289.7053735041076834, -347.2720912057832265 ) ) ;
#50476=CARTESIAN_POINT ( 'NONE',  ( -100.4044040935508662, -282.1289812152826357, -312.4481629479118965 ) ) ;
#50477=CARTESIAN_POINT ( 'NONE',  ( -95.43955505201894596, -290.2026216236845357, -320.8624401911598056 ) ) ;
#50478=CARTESIAN_POINT ( 'NONE',  ( 20.35475171295237828, -287.2552037600265749, -225.6039182061704764 ) ) ;
#50479=DIRECTION ( 'NONE',  ( 0.9951408606192334583, 1.205805641958521361E-17, 0.09846150276129006507 ) ) ;
#50481=CARTESIAN_POINT ( 'NONE',  ( 151.9477299421133125, 206.7868891706451109, -215.8238548150086160 ) ) ;
#50482=CARTESIAN_POINT ( 'NONE',  ( 5.705534526590854583, -59.28686408112852035, -350.9003461107548105 ) ) ;
#50483=CARTESIAN_POINT ( 'NONE',  ( -100.7278341873435323, -277.2482665041739551, -306.9978013252224400 ) ) ;
#50484=CARTESIAN_POINT ( 'NONE',  ( -64.91970509698334979, -278.6035530277573571, -202.4370448132260663 ) ) ;
#50485=CARTESIAN_POINT ( 'NONE',  ( 24.46543051742215269, -274.6085872508367629, -224.4740512538465111 ) ) ;
#50486=CARTESIAN_POINT ( 'NONE',  ( -101.2518121434645622, -256.0555729666142497, -325.2581032958395895 ) ) ;
#50487=CARTESIAN_POINT ( 'NONE',  ( -53.61713600356608822, -278.4221417151254059, -195.6496420831716136 ) ) ;
#50489=CARTESIAN_POINT ( 'NONE',  ( -32.05378935133700935, -281.0052107264659185, -344.8183862846131547 ) ) ;
#50490=CARTESIAN_POINT ( 'NONE',  ( -113.3519438283958038, -298.2856382529115535, -272.4644083437675022 ) ) ;
#50492=CARTESIAN_POINT ( 'NONE',  ( -102.4672627273991310, -291.4952201178479640, -237.1334079464599824 ) ) ;
#50493=CARTESIAN_POINT ( 'NONE',  ( -90.96396670529055939, -288.5179594598225208, -320.6937476754358158 ) ) ;
#50494=CARTESIAN_POINT ( 'NONE',  ( 38.39027062501985199, -276.0355525575665183, -256.9449555593651553 ) ) ;
#50495=CARTESIAN_POINT ( 'NONE',  ( -106.3063850458897832, -272.8704651711901192, -246.4263684708686810 ) ) ;
#50501=CARTESIAN_POINT ( 'NONE',  ( -81.41904606568036229, -281.3779270763285467, -208.9892859210765153 ) ) ;
#50503=CARTESIAN_POINT ( 'NONE',  ( 21.56920778077186895, -282.0223799252533468, -226.7082292495792899 ) ) ;
#50504=CARTESIAN_POINT ( 'NONE',  ( 22.06881807706979259, -282.6693004940840979, -222.9657175083636957 ) ) ;
#50505=CARTESIAN_POINT ( 'NONE',  ( -96.11772671889373498, -283.0000627802093618, -314.0507866341251884 ) ) ;
#50506=CARTESIAN_POINT ( 'NONE',  ( -111.1975082463037836, -280.5162199175214823, -262.3712252633940807 ) ) ;
#50507=CARTESIAN_POINT ( 'NONE',  ( -81.47085739290587014, -271.9196980618636985, -211.2773968101878950 ) ) ;
#50510=CARTESIAN_POINT ( 'NONE',  ( -113.1381988192177630, -279.1969261138105480, -282.9726050801349402 ) ) ;
#50513=CARTESIAN_POINT ( 'NONE',  ( -23.06691515001490345, -275.4478672871723575, -345.4804364020085359 ) ) ;
#50516=CARTESIAN_POINT ( 'NONE',  ( -100.0363718466172713, -285.9686698797094095, -312.2612172582324206 ) ) ;
#50517=CARTESIAN_POINT ( 'NONE',  ( 33.26986962350301269, -293.0022542990965917, -289.5557344872793806 ) ) ;
#50518=CARTESIAN_POINT ( 'NONE',  ( 22.32079750397118900, -287.5527026076826473, -318.8967759123659107 ) ) ;
#50519=CARTESIAN_POINT ( 'NONE',  ( -109.9182901622778701, -282.9808317574454009, -255.8486201017754524 ) ) ;
#50520=CARTESIAN_POINT ( 'NONE',  ( -110.0000325931605687, -283.2806057418363821, -258.6134457570994982 ) ) ;
#50521=CARTESIAN_POINT ( 'NONE',  ( -75.25395888720483129, -287.8047391010647402, -333.9419976261119700 ) ) ;
#50522=CARTESIAN_POINT ( 'NONE',  ( -32.10212280684519470, -284.1896645540531381, -343.5709351837858776 ) ) ;
#50523=CARTESIAN_POINT ( 'NONE',  ( 18.56257173616869949, -272.8551857237717400, -220.2876351543102658 ) ) ;
#50524=CARTESIAN_POINT ( 'NONE',  ( -100.3236513827977632, -283.5246852950218113, -227.3760539709128352 ) ) ;
#50525=CARTESIAN_POINT ( 'NONE',  ( -52.85015154766669809, -297.2509308176731224, -343.7933149615362822 ) ) ;
#50526=CARTESIAN_POINT ( 'NONE',  ( -51.79520111552989192, -283.8676133546560436, -196.5440465423693581 ) ) ;
#50527=CARTESIAN_POINT ( 'NONE',  ( -76.95918794734335222, -280.4487369461126036, -208.7063157858078739 ) ) ;
#50528=CARTESIAN_POINT ( 'NONE',  ( -1.858048916852585331, -288.5212814252029716, -204.0969577940154807 ) ) ;
#50531=CARTESIAN_POINT ( 'NONE',  ( 36.01790000063211039, -295.2415303477548605, -252.2590940450626249 ) ) ;
#50532=CARTESIAN_POINT ( 'NONE',  ( -106.1152682234376385, -276.1589251797670386, -300.4111981247043559 ) ) ;
#50533=CARTESIAN_POINT ( 'NONE',  ( -107.1095149875896482, -290.1634929540900885, -238.0379447303488121 ) ) ;
#50534=CARTESIAN_POINT ( 'NONE',  ( -71.31703719393351548, -293.9083698143986680, -335.8895066952438810 ) ) ;
#50535=CARTESIAN_POINT ( 'NONE',  ( -98.39400186341818255, -277.8025112392520555, -229.3579486722650245 ) ) ;
#50536=CARTESIAN_POINT ( 'NONE',  ( -111.3140475351107455, -270.7397676659972490, -262.0300906769599010 ) ) ;
#50537=CARTESIAN_POINT ( 'NONE',  ( -32.13897964363114568, -293.4342942713402635, -197.0396463758820573 ) ) ;
#50538=CARTESIAN_POINT ( 'NONE',  ( -112.3417001280813849, -275.0519495502701943, -270.3929463913730729 ) ) ;
#50539=CARTESIAN_POINT ( 'NONE',  ( 17.05359745089726076, -292.7741437696052458, -323.9512907131414750 ) ) ;
#50540=CARTESIAN_POINT ( 'NONE',  ( -87.25561993988239351, -291.3615362500224251, -324.7907146433126968 ) ) ;
#50541=CARTESIAN_POINT ( 'NONE',  ( -27.95178620049705742, -290.4095214165646439, -194.9038811779794855 ) ) ;
#50542=CARTESIAN_POINT ( 'NONE',  ( -70.21951838705865612, -290.9194136976122422, -336.2114292482568203 ) ) ;
#50545=CARTESIAN_POINT ( 'NONE',  ( -50.77109552316714769, -290.0308122029234141, -342.3312875913430844 ) ) ;
#50547=CARTESIAN_POINT ( 'NONE',  ( -8.369016963255182517, -289.8862558127065654, -341.2878803557987339 ) ) ;
#50548=CARTESIAN_POINT ( 'NONE',  ( 25.33943359759332736, -280.1348659051067784, -312.1879308853149837 ) ) ;
#50549=CARTESIAN_POINT ( 'NONE',  ( -53.76010863433338471, -280.1804122124978562, -195.0989829989659654 ) ) ;
#50550=CARTESIAN_POINT ( 'NONE',  ( 38.64628956567906215, -281.3739149592637432, -282.7547952723463709 ) ) ;
#50551=CARTESIAN_POINT ( 'NONE',  ( 36.93770649846224785, -285.6863584785522789, -280.8260127570521263 ) ) ;
#50553=CARTESIAN_POINT ( 'NONE',  ( 10.69016339196880061, -280.5200760759428249, -327.0308687734026876 ) ) ;
#50554=CARTESIAN_POINT ( 'NONE',  ( -111.6223074729752938, -282.4142092783552584, -281.0918381816071019 ) ) ;
#50555=CARTESIAN_POINT ( 'NONE',  ( 168.7561003588637334, 230.7615523021927686, -190.5427080440589407 ) ) ;
#50556=CARTESIAN_POINT ( 'NONE',  ( -107.8644361924002766, -277.4057979433205219, -241.2191988774684432 ) ) ;
#50558=CARTESIAN_POINT ( 'NONE',  ( -108.7356630204407537, -283.8305709983785619, -242.2097183485544747 ) ) ;
#50559=CARTESIAN_POINT ( 'NONE',  ( -97.98275434827525032, -273.9237005488904515, -229.3407278936872444 ) ) ;
#50561=CARTESIAN_POINT ( 'NONE',  ( -34.85046563102983441, -293.6840978692334261, -196.6031749020170025 ) ) ;
#50562=CARTESIAN_POINT ( 'NONE',  ( -34.14614178834995784, -275.5168702564121190, -194.0171941846750769 ) ) ;
#50563=CARTESIAN_POINT ( 'NONE',  ( 34.18441814380773280, -275.4127365300766428, -285.0615224604768514 ) ) ;
#50564=CARTESIAN_POINT ( 'NONE',  ( -93.67655316886165906, -297.8643277003683352, -319.8725811360475291 ) ) ;
#50565=CARTESIAN_POINT ( 'NONE',  ( -23.30985349296062736, -289.0443066083440726, -346.1259142551897412 ) ) ;
#50566=CARTESIAN_POINT ( 'NONE',  ( 29.78643164495066742, -280.0876544692137600, -305.0472552696973025 ) ) ;
#50568=CARTESIAN_POINT ( 'NONE',  ( 32.18687852758876744, -292.9599644061058257, -237.1497882578106555 ) ) ;
#50569=CARTESIAN_POINT ( 'NONE',  ( -67.88844043238822223, -290.6998108127315845, -203.7868035206649324 ) ) ;
#50570=CARTESIAN_POINT ( 'NONE',  ( -60.98585703193001706, -293.3587371765879084, -341.5909353593992250 ) ) ;
#50571=ORIENTED_EDGE ( 'NONE', *, *, #39491, .F. ) ;
#50574=CARTESIAN_POINT ( 'NONE',  ( -64.08830546451953580, -291.2012709614912183, -202.3578134652283325 ) ) ;
#50576=CARTESIAN_POINT ( 'NONE',  ( 25.34601139933747760, -287.9050087200863572, -226.0319019468360295 ) ) ;
#50577=CARTESIAN_POINT ( 'NONE',  ( -107.3381139276884824, -270.1608578419545665, -262.4421837807431075 ) ) ;
#50578=CARTESIAN_POINT ( 'NONE',  ( -37.69994709945558498, -294.1152526399672524, -347.1380271246727034 ) ) ;
#50579=CARTESIAN_POINT ( 'NONE',  ( -66.37350456906163743, -284.7395711543567245, -341.1597620802547794 ) ) ;
#50580=CARTESIAN_POINT ( 'NONE',  ( -108.0281295831141222, -284.6261586026583927, -252.1284907602799876 ) ) ;
#50581=CARTESIAN_POINT ( 'NONE',  ( 32.76367154741866727, -277.3707948775800674, -293.0755322310818087 ) ) ;
#50582=CARTESIAN_POINT ( 'NONE',  ( -3.615561839231120178, -292.6249790993928173, -336.9666782701792727 ) ) ;
#50583=CARTESIAN_POINT ( 'NONE',  ( -35.60466796355051144, -296.7902389358005735, -344.3667378590021144 ) ) ;
#50584=AXIS2_PLACEMENT_3D ( 'NONE', #49757, #64006, #14733 ) ;
#50585=CARTESIAN_POINT ( 'NONE',  ( 30.64003728721610642, -274.7173237397886965, -298.1660121536711472 ) ) ;
#50588=CARTESIAN_POINT ( 'NONE',  ( 37.76235922683074619, -293.4308532070033948, -287.3062319609697397 ) ) ;
#50589=CARTESIAN_POINT ( 'NONE',  ( 37.12011636808607307, -289.4449720439729390, -268.2476503550930715 ) ) ;
#50590=CARTESIAN_POINT ( 'NONE',  ( 200.9868139007817263, 294.2258809633341343, -54.00000000000627409 ) ) ;
#50591=CARTESIAN_POINT ( 'NONE',  ( 75.80595655901278462, -300.5172811257933176, -193.6499684678605036 ) ) ;
#50592=CARTESIAN_POINT ( 'NONE',  ( -57.43035015493347828, -286.4374757898834218, -200.0208854630392068 ) ) ;
#50594=CARTESIAN_POINT ( 'NONE',  ( -61.96078719651509203, -278.7986436637582983, -197.5952210541718728 ) ) ;
#50595=CARTESIAN_POINT ( 'NONE',  ( -53.26003357299727980, -295.9024005646747923, -345.6480237536758864 ) ) ;
#50596=CARTESIAN_POINT ( 'NONE',  ( -51.47843674278839643, -287.3706754109274470, -344.7953718971581338 ) ) ;
#50598=CARTESIAN_POINT ( 'NONE',  ( -94.63300086554374957, -296.1874574772651272, -321.7952590677210765 ) ) ;
#50599=CARTESIAN_POINT ( 'NONE',  ( 6.685613656262284543, -293.0032402247386472, -212.1057909504669112 ) ) ;
#50600=CARTESIAN_POINT ( 'NONE',  ( 129.4467878515196162, -299.5541904835127980, -195.3611179825600175 ) ) ;
#50603=CARTESIAN_POINT ( 'NONE',  ( -30.96129520394098478, -287.6514862100369783, -194.3084914561176504 ) ) ;
#50604=CARTESIAN_POINT ( 'NONE',  ( -2.659677404128736544, -292.1237833571632336, -342.4524372437778652 ) ) ;
#50607=CARTESIAN_POINT ( 'NONE',  ( -28.22883870408087503, -279.5133601797209053, -193.9513684470461783 ) ) ;
#50608=CARTESIAN_POINT ( 'NONE',  ( -29.22100949224067179, -284.9493176896522186, -344.8043067740237575 ) ) ;
#50610=CARTESIAN_POINT ( 'NONE',  ( -91.47267292630989743, -283.8744249994660436, -216.4311256210886540 ) ) ;
#50611=CARTESIAN_POINT ( 'NONE',  ( 11.03284419091577995, -286.4567719829759653, -327.0085594551189274 ) ) ;
#50612=CARTESIAN_POINT ( 'NONE',  ( 35.70122412836058601, -277.6693433025096169, -290.5350726345512840 ) ) ;
#50613=CARTESIAN_POINT ( 'NONE',  ( -102.5901131178605681, -297.4916430258418814, -237.3754689325374443 ) ) ;
#50615=CARTESIAN_POINT ( 'NONE',  ( 33.58828221144553794, -292.4899956675226917, -289.6490160998978354 ) ) ;
#50616=CARTESIAN_POINT ( 'NONE',  ( -100.8118069179065799, -279.0460627205999913, -234.2980406861314009 ) ) ;
#50617=CARTESIAN_POINT ( 'NONE',  ( -99.55011862251508603, -278.4305625841293477, -231.8717899216632929 ) ) ;
#50618=CARTESIAN_POINT ( 'NONE',  ( -36.95515232414381046, -275.1365832126898567, -193.6582033488697050 ) ) ;
#50619=CARTESIAN_POINT ( 'NONE',  ( -112.4076225778830889, -277.1543271996079625, -285.6941421875354763 ) ) ;
#50620=CARTESIAN_POINT ( 'NONE',  ( 200.9738562182569694, 294.2969822784109510, -54.00000000000292744 ) ) ;
#50621=CARTESIAN_POINT ( 'NONE',  ( -98.63077282400308832, -298.5892371604248865, -224.7075320890699572 ) ) ;
#50625=CARTESIAN_POINT ( 'NONE',  ( -4.468222450009211144, -287.5756352958367756, -204.8358515586194812 ) ) ;
#50626=CARTESIAN_POINT ( 'NONE',  ( -36.59816230708373297, -287.8214984955697560, -194.3652189482223491 ) ) ;
#50627=CARTESIAN_POINT ( 'NONE',  ( 32.40837719230589897, -287.1923481898029422, -292.4114728223817679 ) ) ;
#50628=CARTESIAN_POINT ( 'NONE',  ( -112.1607808670383690, -283.8346397242334547, -288.3510100265839924 ) ) ;
#50629=CARTESIAN_POINT ( 'NONE',  ( -108.7414440732028851, -277.1964146775194422, -251.6429237998689814 ) ) ;
#50630=CARTESIAN_POINT ( 'NONE',  ( -103.3473028478311448, -286.8666932402496741, -236.3886896451549546 ) ) ;
#50631=CARTESIAN_POINT ( 'NONE',  ( 22.36239618090853654, -280.6309400931646110, -313.5814276142867243 ) ) ;
#50632=CARTESIAN_POINT ( 'NONE',  ( -35.08583151312780046, -278.3384105242751616, -343.8196405377458404 ) ) ;
#50633=CARTESIAN_POINT ( 'NONE',  ( 19.89980603403492054, -275.4039490821534173, -224.9384763172944020 ) ) ;
#50634=CARTESIAN_POINT ( 'NONE',  ( -12.36775838504746261, -287.5294454251916818, -342.8343117162604017 ) ) ;
#50635=CARTESIAN_POINT ( 'NONE',  ( -92.31106530986541259, -284.6169264535692491, -324.0502948419393192 ) ) ;
#50636=CARTESIAN_POINT ( 'NONE',  ( 36.42148273580804840, -282.3212365474557828, -292.4195444758761369 ) ) ;
#50637=ORIENTED_EDGE ( 'NONE', *, *, #80735, .T. ) ;
#50638=ORIENTED_EDGE ( 'NONE', *, *, #59261, .T. ) ;
#50640=CARTESIAN_POINT ( 'NONE',  ( -73.81161595310983614, -291.3914379336896445, -336.7856464069825506 ) ) ;
#50641=CARTESIAN_POINT ( 'NONE',  ( -112.6508663995820996, -289.0663228429464198, -283.9195570222651668 ) ) ;
#50643=CARTESIAN_POINT ( 'NONE',  ( -83.32906147637478966, -272.4625435929074797, -213.3648808822834440 ) ) ;
#50644=CARTESIAN_POINT ( 'NONE',  ( 30.81243232566732715, -292.4393703750646409, -234.6328833485093242 ) ) ;
#50645=CARTESIAN_POINT ( 'NONE',  ( -106.6915217162919021, -288.7031856193524959, -295.2872086778048129 ) ) ;
#50646=CARTESIAN_POINT ( 'NONE',  ( 5.102856127595141622, -290.8742407376810206, -209.6646775858870626 ) ) ;
#50648=CARTESIAN_POINT ( 'NONE',  ( 34.40205780873399277, -288.9611997452870469, -285.9108841845203415 ) ) ;
#50649=CARTESIAN_POINT ( 'NONE',  ( -37.37352853689063892, -294.5519495502701943, -195.3611179825600175 ) ) ;
#50650=CARTESIAN_POINT ( 'NONE',  ( 34.47777196055003657, -289.8312778949887161, -292.0151259681339297 ) ) ;
#50651=CARTESIAN_POINT ( 'NONE',  ( -109.0409849057111842, -288.2595304861441718, -293.0977176048550632 ) ) ;
#50652=CARTESIAN_POINT ( 'NONE',  ( -20.80378870078060771, -294.2644622551550810, -197.1545517989554526 ) ) ;
#50653=CARTESIAN_POINT ( 'NONE',  ( -108.6516683530374081, -285.2733919744090940, -287.0981029724775340 ) ) ;
#50654=CARTESIAN_POINT ( 'NONE',  ( -14.44962477803068879, -294.3482656831655504, -198.7105233637303741 ) ) ;
#50657=CARTESIAN_POINT ( 'NONE',  ( -77.97628912913027932, -275.4888363911822466, -206.9006028719965968 ) ) ;
#50658=AXIS2_PLACEMENT_3D ( 'NONE', #81419, #16569, #8527 ) ;
#50659=CARTESIAN_POINT ( 'NONE',  ( 21.93678298466754484, -281.3481135854267450, -313.2621999167705553 ) ) ;
#50660=CARTESIAN_POINT ( 'NONE',  ( -62.22157222968028378, -281.3754123324009129, -341.1688601846573761 ) ) ;
#50661=CARTESIAN_POINT ( 'NONE',  ( -98.15294642187133434, -295.1210667941875272, -317.3308012409939920 ) ) ;
#50662=CARTESIAN_POINT ( 'NONE',  ( -62.35131544482404564, -271.9621581253859404, -200.7012790894118837 ) ) ;
#50663=CARTESIAN_POINT ( 'NONE',  ( -110.1787384329058881, -276.4332307719452615, -285.7260147363729743 ) ) ;
#50664=CARTESIAN_POINT ( 'NONE',  ( -110.5431099916445419, -297.9602667386751591, -263.2686088970505125 ) ) ;
#50665=CARTESIAN_POINT ( 'NONE',  ( 12.76929281322739840, -295.7621540178243436, -324.3221933111759654 ) ) ;
#50667=CARTESIAN_POINT ( 'NONE',  ( 18.10147307412642448, -295.0334770871054957, -318.1154958204226659 ) ) ;
#50669=CARTESIAN_POINT ( 'NONE',  ( -21.30880671319026476, -284.2769166707300883, -196.7312794081399545 ) ) ;
#50670=CARTESIAN_POINT ( 'NONE',  ( -82.35981002355005387, -295.6861283191742586, -327.8918156675024420 ) ) ;
#50671=CARTESIAN_POINT ( 'NONE',  ( -97.58040072872390169, -285.1942720901694202, -222.3996860820615780 ) ) ;
#50672=CARTESIAN_POINT ( 'NONE',  ( 31.66658393045714703, -287.6587045706564822, -304.5929185477433521 ) ) ;
#50673=CARTESIAN_POINT ( 'NONE',  ( 10.02857173849627159, -290.7060881060497763, -212.3621536886592196 ) ) ;
#50674=CARTESIAN_POINT ( 'NONE',  ( -84.45983355236950274, -278.6195861815552917, -209.5974960875428508 ) ) ;
#50675=CARTESIAN_POINT ( 'NONE',  ( -69.91165696735023971, -280.9809262143061233, -337.9199732462171255 ) ) ;
#50677=CARTESIAN_POINT ( 'NONE',  ( 36.07798791811234906, -286.3202451397177697, -268.3166277008521092 ) ) ;
#50678=CARTESIAN_POINT ( 'NONE',  ( -74.29050612810728182, -288.4518254657351690, -337.5793730325070783 ) ) ;
#50681=CARTESIAN_POINT ( 'NONE',  ( -103.4761154527324152, -297.7117424962871723, -303.2283240874078274 ) ) ;
#50682=CARTESIAN_POINT ( 'NONE',  ( 30.19247539282088155, -282.5109778659253834, -234.5028554381205481 ) ) ;
#50683=CARTESIAN_POINT ( 'NONE',  ( -94.31070658806939377, -295.2538411404576664, -220.9584413619001566 ) ) ;
#50684=CARTESIAN_POINT ( 'NONE',  ( 34.25056937097342313, -281.4092718712283272, -284.7988101712308548 ) ) ;
#50685=CARTESIAN_POINT ( 'NONE',  ( 11.19995734515881658, -294.5679551348339373, -330.2019603090411124 ) ) ;
#50686=CARTESIAN_POINT ( 'NONE',  ( 19.22528429898121516, -284.9398263185986480, -220.1890358981652298 ) ) ;
#50687=CARTESIAN_POINT ( 'NONE',  ( -40.93863963214825219, -282.0070757780899271, -195.4345638159099678 ) ) ;
#50688=CARTESIAN_POINT ( 'NONE',  ( -110.6197293275990745, -295.5965144270879250, -271.4547072078576093 ) ) ;
#50689=ORIENTED_EDGE ( 'NONE', *, *, #37043, .T. ) ;
#50691=CARTESIAN_POINT ( 'NONE',  ( 6.579800234881638232, -284.4316580313373493, -330.7163050484019209 ) ) ;
#50693=CARTESIAN_POINT ( 'NONE',  ( -69.91165696735023971, -292.9809262143061801, -337.9199732462171255 ) ) ;
#50694=CARTESIAN_POINT ( 'NONE',  ( 35.90560846230874859, -275.0417417524660095, -293.5772891723465818 ) ) ;
#50695=CARTESIAN_POINT ( 'NONE',  ( -2.437568201589315198, -292.3608657699249420, -206.2321693465572139 ) ) ;
#50696=CARTESIAN_POINT ( 'NONE',  ( 28.39116024668721749, -282.6228366929426556, -236.9328830591988151 ) ) ;
#50697=CARTESIAN_POINT ( 'NONE',  ( 12.06716573470712461, -276.3526501189858777, -215.4725813228913580 ) ) ;
#50698=CARTESIAN_POINT ( 'NONE',  ( -70.10745526814440609, -285.0766877169907616, -339.1711087785158725 ) ) ;
#50699=CARTESIAN_POINT ( 'NONE',  ( 27.19694827246567925, -280.8214523779101910, -305.3167093293772041 ) ) ;
#50700=CARTESIAN_POINT ( 'NONE',  ( -103.6125706703960105, -280.0867013966838499, -305.4776719624892394 ) ) ;
#50701=CARTESIAN_POINT ( 'NONE',  ( -31.90953307493142432, -298.1184045043421520, -193.3611177971762629 ) ) ;
#50702=CARTESIAN_POINT ( 'NONE',  ( 39.70736890770487548, -275.3956356849034819, -271.1737616800800197 ) ) ;
#50703=CARTESIAN_POINT ( 'NONE',  ( 35.18383762991108910, -295.6899563490876517, -287.1911619270002802 ) ) ;
#50706=CARTESIAN_POINT ( 'NONE',  ( 18.60137137966103893, -292.3984765948715676, -321.5323030299247762 ) ) ;
#50707=CARTESIAN_POINT ( 'NONE',  ( -8.941124562624166217, -273.9414469537405807, -202.9915158831300630 ) ) ;
#50709=CARTESIAN_POINT ( 'NONE',  ( -61.48770697605829127, -293.2643344410296322, -197.9198407806392197 ) ) ;
#50710=CARTESIAN_POINT ( 'NONE',  ( -37.30987171927208124, -285.5519495502701943, -345.3611179825600175 ) ) ;
#50711=CARTESIAN_POINT ( 'NONE',  ( -6.063184400527456219, -293.6592104890349901, -200.4207782973604992 ) ) ;
#50713=CARTESIAN_POINT ( 'NONE',  ( -64.46213936458900662, -291.4069716188662369, -340.1626961888671303 ) ) ;
#50714=CARTESIAN_POINT ( 'NONE',  ( -106.9830185894094967, -276.1947112019400379, -297.7493487986541254 ) ) ;
#50715=CARTESIAN_POINT ( 'NONE',  ( -46.05280787783291885, -279.0835004935420329, -344.3412935959492529 ) ) ;
#50716=CARTESIAN_POINT ( 'NONE',  ( 33.71419598572568788, -291.9203614786669618, -292.5506160771714690 ) ) ;
#50717=CARTESIAN_POINT ( 'NONE',  ( 36.00213520313938176, -283.6542354542758062, -289.3607838231470737 ) ) ;
#50720=CARTESIAN_POINT ( 'NONE',  ( -86.94631203140275488, -283.4320030987371979, -324.0163969824542960 ) ) ;
#50721=CARTESIAN_POINT ( 'NONE',  ( -69.84393356210931358, -280.7138156454767568, -200.8838649187784142 ) ) ;
#50722=CARTESIAN_POINT ( 'NONE',  ( -107.5559965380076335, -283.7410510017319325, -239.6023945491425309 ) ) ;
#50723=CARTESIAN_POINT ( 'NONE',  ( -113.5311806594003485, -279.3704599795316881, -280.1613874285964698 ) ) ;
#50725=CARTESIAN_POINT ( 'NONE',  ( 38.03963286382045084, -276.9216938620741644, -258.4295648329849087 ) ) ;
#50726=CARTESIAN_POINT ( 'NONE',  ( -92.08974858914540107, -281.6948066931272479, -226.7417163044926838 ) ) ;
#50729=CARTESIAN_POINT ( 'NONE',  ( -80.91001088341863579, -299.4608118134544270, -209.3135713977811179 ) ) ;
#50730=CARTESIAN_POINT ( 'NONE',  ( -110.9114014661921601, -276.4084302246379821, -283.0600420439504887 ) ) ;
#50731=CARTESIAN_POINT ( 'NONE',  ( -90.09873469613977193, -293.0793954024132972, -215.6010580598285173 ) ) ;
#50732=CARTESIAN_POINT ( 'NONE',  ( 26.32740895562920258, -292.4085421475554654, -234.3392601364453753 ) ) ;
#50733=CARTESIAN_POINT ( 'NONE',  ( -106.4609867064203712, -289.6241382072789179, -304.2764854710000009 ) ) ;
#50735=CARTESIAN_POINT ( 'NONE',  ( -2.254333340841217836, -293.1716730803213977, -338.2395607049411410 ) ) ;
#50736=CARTESIAN_POINT ( 'NONE',  ( -52.23063916488089120, -284.2582001884280203, -198.0786172828219946 ) ) ;
#50737=CARTESIAN_POINT ( 'NONE',  ( -47.18124592499035685, -293.7862433429260705, -196.7808976971628567 ) ) ;
#50738=CARTESIAN_POINT ( 'NONE',  ( -38.61767950440530939, -284.5157764704475198, -196.6662290483114077 ) ) ;
#50739=CARTESIAN_POINT ( 'NONE',  ( -76.37494997296566623, -284.9008398512291365, -332.6920662321321629 ) ) ;
#50741=CARTESIAN_POINT ( 'NONE',  ( -102.0963135441440244, -290.9502177219982855, -311.6858505583379610 ) ) ;
#50742=CARTESIAN_POINT ( 'NONE',  ( -46.47035794410771103, -280.4256689822112207, -197.8209659284459860 ) ) ;
#50743=CARTESIAN_POINT ( 'NONE',  ( 38.42154991089551430, -292.4892729283961330, -281.6721153807094424 ) ) ;
#50744=CARTESIAN_POINT ( 'NONE',  ( -12.26674238007786499, -289.5370301748904467, -343.0488609188486748 ) ) ;
#50745=CARTESIAN_POINT ( 'NONE',  ( 31.63503424509521977, -288.4842000853440140, -304.5655557062778485 ) ) ;
#50746=CARTESIAN_POINT ( 'NONE',  ( -62.56486507424283161, -285.8814005000231759, -201.8032535258574285 ) ) ;
#50748=CARTESIAN_POINT ( 'NONE',  ( 16.69743347904245923, -296.1541367301069272, -323.5401653480811319 ) ) ;
#50749=CARTESIAN_POINT ( 'NONE',  ( -70.60867867298426859, -294.1664226859015798, -339.2711560559325221 ) ) ;
#50750=CARTESIAN_POINT ( 'NONE',  ( -107.4489064527324160, -277.8903522662457135, -249.1859421936339913 ) ) ;
#50751=CARTESIAN_POINT ( 'NONE',  ( -52.52733496536654911, -273.3704382455338759, -194.8817693074799422 ) ) ;
#50752=CARTESIAN_POINT ( 'NONE',  ( -4.040505564498671376, -293.0846749569743679, -336.1151760675631408 ) ) ;
#50753=CARTESIAN_POINT ( 'NONE',  ( 33.06900828615941634, -277.6107754190001060, -293.1713383672232567 ) ) ;
#50754=CARTESIAN_POINT ( 'NONE',  ( -95.56702226212388496, -271.3308114531208162, -224.3103053257931663 ) ) ;
#50755=CARTESIAN_POINT ( 'NONE',  ( 6.903457906644599795, -293.8748944755399748, -211.7992148872943119 ) ) ;
#50756=CARTESIAN_POINT ( 'NONE',  ( -36.98027337336755238, -296.1271627618154412, -343.6818172421015447 ) ) ;
#50758=CARTESIAN_POINT ( 'NONE',  ( -106.0857824942959695, -294.9508387485374783, -239.8305610484518695 ) ) ;
#50759=CARTESIAN_POINT ( 'NONE',  ( -57.37117490026938071, -298.4517819281128936, -196.0621710246494160 ) ) ;
#50760=CARTESIAN_POINT ( 'NONE',  ( -64.04190175609727476, -275.7040825153271157, -200.2608782645664007 ) ) ;
#50761=CARTESIAN_POINT ( 'NONE',  ( -94.27967900351522701, -290.8439995039550467, -316.4205905208636977 ) ) ;
#50762=CARTESIAN_POINT ( 'NONE',  ( -38.33832540295010460, -295.3982680791398252, -343.3754605799539377 ) ) ;
#50763=CARTESIAN_POINT ( 'NONE',  ( -95.76287256738045528, -279.8791551393359214, -317.9772558348826124 ) ) ;
#50764=CARTESIAN_POINT ( 'NONE',  ( -74.75207895309200978, -278.2497119911328127, -203.6246075156549864 ) ) ;
#50766=CARTESIAN_POINT ( 'NONE',  ( -0.4316617390987354530, -281.9233504309728460, -337.8368537223751105 ) ) ;
#50767=CARTESIAN_POINT ( 'NONE',  ( 37.80429224485347106, -275.1059065389146667, -286.7441482194013815 ) ) ;
#50768=CARTESIAN_POINT ( 'NONE',  ( -69.60491725636561000, -278.0344500815253923, -201.3140957296970157 ) ) ;
#50769=CARTESIAN_POINT ( 'NONE',  ( 0.4742104381092190901, -278.5542552046782134, -205.3404340612911767 ) ) ;
#50770=CARTESIAN_POINT ( 'NONE',  ( -96.48730095058181178, -295.8445424001401420, -226.7160153247493497 ) ) ;
#50771=CARTESIAN_POINT ( 'NONE',  ( 36.98253148569139626, -277.6860573295540462, -280.7773555883468930 ) ) ;
#50773=CARTESIAN_POINT ( 'NONE',  ( -70.15814442175897625, -289.6420187720629542, -202.5268508920531758 ) ) ;
#50774=CARTESIAN_POINT ( 'NONE',  ( -82.85264511769260309, -289.6556945937999785, -332.4719373794459329 ) ) ;
#50775=CARTESIAN_POINT ( 'NONE',  ( 35.50210460976308724, -277.3146272681639743, -251.8190430911533326 ) ) ;
#50776=CARTESIAN_POINT ( 'NONE',  ( -83.04413536489295211, -295.4252800982309282, -211.0391032491959606 ) ) ;
#50777=CARTESIAN_POINT ( 'NONE',  ( -73.52791007730634476, -284.7820242808957119, -202.5178488926247269 ) ) ;
#50779=CARTESIAN_POINT ( 'NONE',  ( -97.44968100573896663, -281.9391343560257042, -315.2379391244991211 ) ) ;
#50782=CARTESIAN_POINT ( 'NONE',  ( -17.30956238412722570, -291.1112886620433642, -199.6977270563631635 ) ) ;
#50783=CARTESIAN_POINT ( 'NONE',  ( -105.7263268552588897, -283.0745539338489607, -241.3429665046753598 ) ) ;
#50786=CARTESIAN_POINT ( 'NONE',  ( -8.947307919121019637, -290.4232240490219965, -200.8885671734395260 ) ) ;
#50787=CARTESIAN_POINT ( 'NONE',  ( -63.69093037313236749, -281.8694044047651346, -341.9741462506141829 ) ) ;
#50788=CARTESIAN_POINT ( 'NONE',  ( -94.20959947682335667, -279.4924573109801145, -317.4179434772631225 ) ) ;
#50789=CARTESIAN_POINT ( 'NONE',  ( -108.6644279661540082, -286.1149502404304030, -242.2690279585470989 ) ) ;
#50790=CARTESIAN_POINT ( 'NONE',  ( -57.39438582579897030, -285.7861674244165897, -200.1166974895409396 ) ) ;
#50791=CARTESIAN_POINT ( 'NONE',  ( -109.8636942137055712, -279.8130446852018167, -282.9229001058603785 ) ) ;
#50792=CARTESIAN_POINT ( 'NONE',  ( -83.54761871295198716, -280.2026885517768164, -213.5715159063096849 ) ) ;
#50793=CARTESIAN_POINT ( 'NONE',  ( -111.1636761064662977, -286.3786482079773918, -283.8864502161146106 ) ) ;
#50795=CARTESIAN_POINT ( 'NONE',  ( -30.48245140136254605, -297.9691305585425880, -193.3613054221744960 ) ) ;
#50796=CARTESIAN_POINT ( 'NONE',  ( -18.02406063249808099, -290.7819362710985160, -342.5167353693213954 ) ) ;
#50798=CARTESIAN_POINT ( 'NONE',  ( -72.08107566293803359, -288.1233781216987495, -198.2974183793908196 ) ) ;
#50800=CARTESIAN_POINT ( 'NONE',  ( 33.72419005074169718, -291.5983825486693490, -242.7182971222643744 ) ) ;
#50801=CARTESIAN_POINT ( 'NONE',  ( 36.37336663727020181, -289.0450043253065928, -268.2736880560483996 ) ) ;
#50802=CARTESIAN_POINT ( 'NONE',  ( 34.08569886428286821, -283.0590458122868540, -250.9193692827377333 ) ) ;
#50803=CARTESIAN_POINT ( 'NONE',  ( 36.22210640171046947, -289.2389047819781354, -291.0724606052908712 ) ) ;
#50804=CARTESIAN_POINT ( 'NONE',  ( 38.19086499478468255, -289.0245762020866209, -282.8544962804359670 ) ) ;
#50805=CARTESIAN_POINT ( 'NONE',  ( -94.05523728357189839, -285.8714485915557475, -319.4578920669638364 ) ) ;
#50806=CARTESIAN_POINT ( 'NONE',  ( -97.92759369401956349, -278.0835456849674188, -317.8832129001044677 ) ) ;
#50807=ORIENTED_EDGE ( 'NONE', *, *, #43456, .F. ) ;
#50808=CARTESIAN_POINT ( 'NONE',  ( -5.138864125718958675, -292.7114819676794468, -338.7294772909415315 ) ) ;
#50809=CARTESIAN_POINT ( 'NONE',  ( 37.67798015011608470, -281.1678237666186533, -252.9524576551812061 ) ) ;
#50810=CARTESIAN_POINT ( 'NONE',  ( -83.98476371509421767, -275.2637606583527941, -212.6091474824507941 ) ) ;
#50813=CARTESIAN_POINT ( 'NONE',  ( -69.85430415644619018, -291.9805209788416391, -337.9475929042657754 ) ) ;
#50814=CARTESIAN_POINT ( 'NONE',  ( -57.82659860805578234, -272.0311321130779447, -197.1330511315456704 ) ) ;
#50816=CARTESIAN_POINT ( 'NONE',  ( -14.28351504931984017, -279.8668964921849351, -200.9800866251921434 ) ) ;
#50817=CARTESIAN_POINT ( 'NONE',  ( -11.98307774365967937, -277.9345030618075612, -342.7005696370524106 ) ) ;
#50818=CARTESIAN_POINT ( 'NONE',  ( -63.30420472870662252, -299.1325798379118055, -201.4499332045505753 ) ) ;
#50819=CARTESIAN_POINT ( 'NONE',  ( -65.17807595261378140, -282.4658927849517340, -341.9151730905829254 ) ) ;
#50820=CARTESIAN_POINT ( 'NONE',  ( -93.16140682518464189, -291.6280854516674594, -319.0394720045267150 ) ) ;
#50821=CARTESIAN_POINT ( 'NONE',  ( -99.36935526849525502, -298.6665412092883116, -225.9170210588498833 ) ) ;
#50822=CARTESIAN_POINT ( 'NONE',  ( -14.96982002085689700, -299.5314604421131435, -193.7537215998492570 ) ) ;
#50823=CARTESIAN_POINT ( 'NONE',  ( 34.10455622380240470, -295.8400433987417841, -292.6200685462527531 ) ) ;
#50824=CARTESIAN_POINT ( 'NONE',  ( -43.09875214564075208, -281.1247050262921334, -345.0240214393301699 ) ) ;
#50825=CARTESIAN_POINT ( 'NONE',  ( -79.57926831555381852, -291.1653667752359524, -205.9411111316073004 ) ) ;
#50826=CARTESIAN_POINT ( 'NONE',  ( -36.69709821686532081, -272.0803988026510751, -195.7064017538280041 ) ) ;
#50827=CARTESIAN_POINT ( 'NONE',  ( -65.59982650302146112, -287.2888733781849169, -199.5804589851779269 ) ) ;
#50828=CARTESIAN_POINT ( 'NONE',  ( -72.51921916857611450, -288.4498391899437024, -334.6788311593118692 ) ) ;
#50829=CARTESIAN_POINT ( 'NONE',  ( -82.59061302912155611, -220.2773766338590633, -352.3396032511032558 ) ) ;
#50831=CARTESIAN_POINT ( 'NONE',  ( -96.11393532843437981, -289.7887860191331697, -221.5102719404187610 ) ) ;
#50832=CARTESIAN_POINT ( 'NONE',  ( -42.66969263814385727, -288.7877950589927423, -343.2382426531012811 ) ) ;
#50834=CARTESIAN_POINT ( 'NONE',  ( -15.51464989385819848, -287.4077357868389413, -196.7867540621706723 ) ) ;
#50835=CARTESIAN_POINT ( 'NONE',  ( 0.8861114934221715478, -276.8604751478663957, -332.6356594363435306 ) ) ;
#50837=CARTESIAN_POINT ( 'NONE',  ( 33.04616037973165987, -292.0829378409865171, -239.9137600995213120 ) ) ;
#50838=CARTESIAN_POINT ( 'NONE',  ( -112.4237661626760314, -284.9955161575650209, -286.9742497502320475 ) ) ;
#50839=CARTESIAN_POINT ( 'NONE',  ( 6.542239102787454463, -283.9881232360132230, -332.8509590032899723 ) ) ;
#50840=CARTESIAN_POINT ( 'NONE',  ( -76.74342330689559333, -283.8973773675526218, -336.5534597473719032 ) ) ;
#50841=CARTESIAN_POINT ( 'NONE',  ( 22.12824792924733330, -281.2936889681581647, -227.9888066828895319 ) ) ;
#50842=CARTESIAN_POINT ( 'NONE',  ( -112.4251224187018465, -271.4489424832871691, -296.3911511650422881 ) ) ;
#50843=CARTESIAN_POINT ( 'NONE',  ( 200.9643288768799607, 293.5986974642797236, -83.07126776150519731 ) ) ;
#50844=CARTESIAN_POINT ( 'NONE',  ( -71.24468398583613293, -195.3788060869234755, -356.9306778524392030 ) ) ;
#50845=CARTESIAN_POINT ( 'NONE',  ( -64.61951886301119430, -272.8838609646115856, -202.4615110291326801 ) ) ;
#50846=CARTESIAN_POINT ( 'NONE',  ( -3.261686557078808946, -294.1218671727963283, -339.3545440673736948 ) ) ;
#50847=CARTESIAN_POINT ( 'NONE',  ( -54.50862104011823561, -170.0898157090607299, -361.0194490113770485 ) ) ;
#50848=CARTESIAN_POINT ( 'NONE',  ( -55.20214254111591146, -272.5118857717246783, -195.9682227019258391 ) ) ;
#50849=CARTESIAN_POINT ( 'NONE',  ( -111.3282006056732314, -298.3260144464038035, -277.0338532795914261 ) ) ;
#50850=CARTESIAN_POINT ( 'NONE',  ( 34.18643073227132589, -288.6454207686007294, -253.4257274208140416 ) ) ;
#50851=VERTEX_POINT ( 'NONE', #38427 ) ;
#50852=CARTESIAN_POINT ( 'NONE',  ( -22.13240718812397034, -295.8031420716584989, -345.6040420389776955 ) ) ;
#50854=CARTESIAN_POINT ( 'NONE',  ( -6.996661576786002534, -286.9537537187511589, -203.8856087334964968 ) ) ;
#50855=CARTESIAN_POINT ( 'NONE',  ( -73.78580049746170744, -272.5005970861380433, -202.8237949150263262 ) ) ;
#50856=CARTESIAN_POINT ( 'NONE',  ( 37.30557950669378187, -294.5839869356539680, -288.6354919991429142 ) ) ;
#50857=CARTESIAN_POINT ( 'NONE',  ( -99.95476595430773159, -296.4507365763180928, -315.1624850692325026 ) ) ;
#50858=CARTESIAN_POINT ( 'NONE',  ( -77.25693139233162299, -291.6670159748055653, -209.2401369890033038 ) ) ;
#50860=CARTESIAN_POINT ( 'NONE',  ( -65.70971136271141688, -275.6041903581665338, -200.3145743447263953 ) ) ;
#50861=CARTESIAN_POINT ( 'NONE',  ( 24.17023763975591777, -273.7369336271359543, -224.7070904316422570 ) ) ;
#50863=CARTESIAN_POINT ( 'NONE',  ( -103.5560301905008629, -277.5477989348951269, -309.6471017368729122 ) ) ;
#50864=CARTESIAN_POINT ( 'NONE',  ( 28.58498052853238391, -273.5067583028380227, -237.1931637098956855 ) ) ;
#50865=CARTESIAN_POINT ( 'NONE',  ( -110.4982612007245990, -273.7035134877704081, -264.9040783715561247 ) ) ;
#50866=CARTESIAN_POINT ( 'NONE',  ( 7.465445680261517225, -275.6219831932619968, -212.4324710806345422 ) ) ;
#50867=CARTESIAN_POINT ( 'NONE',  ( 97.40392376569691635, -301.3126994743653313, -194.1250687223027001 ) ) ;
#50868=CARTESIAN_POINT ( 'NONE',  ( 36.29292874655875778, -273.7776425915074014, -286.4321930518889872 ) ) ;
#50869=CARTESIAN_POINT ( 'NONE',  ( -45.09330768877237006, -295.8041826238767271, -343.1014528061047031 ) ) ;
#50870=CARTESIAN_POINT ( 'NONE',  ( 34.79767957394593481, -291.9366630849207240, -255.8254785111904823 ) ) ;
#50872=CARTESIAN_POINT ( 'NONE',  ( -108.4581650032118603, -279.4179430854298403, -241.0017016610278802 ) ) ;
#50873=CARTESIAN_POINT ( 'NONE',  ( 35.02022914173060286, -275.5917875855570287, -260.7303757030665565 ) ) ;
#50874=CARTESIAN_POINT ( 'NONE',  ( -95.43107978121291524, -283.9138448870438083, -220.4929019986416847 ) ) ;
#50875=CARTESIAN_POINT ( 'NONE',  ( -112.5315993034798367, -298.5256188962545139, -272.4450014759427745 ) ) ;
#50877=CARTESIAN_POINT ( 'NONE',  ( -9.422326905928947838, -285.6237696785283902, -202.7228032636003263 ) ) ;
#50878=CARTESIAN_POINT ( 'NONE',  ( -109.4789013923819709, -276.5758298443051899, -286.9762884760010024 ) ) ;
#50879=CARTESIAN_POINT ( 'NONE',  ( -73.14442872080606151, -276.1113507012303216, -334.6682263215733428 ) ) ;
#50880=CARTESIAN_POINT ( 'NONE',  ( -22.79041941096711810, -284.8662421930104074, -343.9882306272708661 ) ) ;
#50881=CARTESIAN_POINT ( 'NONE',  ( 16.83455455260827804, -277.4638744020754757, -319.8981872453594519 ) ) ;
#50883=CARTESIAN_POINT ( 'NONE',  ( 26.27401679483157437, -273.3946727148648392, -228.4149503928773299 ) ) ;
#50884=CARTESIAN_POINT ( 'NONE',  ( -16.61970088106266275, -274.9783366215162346, -200.2049044040248020 ) ) ;
#50885=CARTESIAN_POINT ( 'NONE',  ( -38.17574050438641109, -282.0418783454302911, -195.1990743197127927 ) ) ;
#50886=CARTESIAN_POINT ( 'NONE',  ( 144.2857639756989272, -299.5541904835127980, -195.3611179825600175 ) ) ;
#50887=CARTESIAN_POINT ( 'NONE',  ( 29.10818525265068146, -289.9476976713093563, -306.4390229381738777 ) ) ;
#50888=CARTESIAN_POINT ( 'NONE',  ( 7.065082734878200377, -292.4477149551959769, -330.8652190956427148 ) ) ;
#50890=CARTESIAN_POINT ( 'NONE',  ( -96.66962088441499645, -271.8413216895959863, -226.9010071387581036 ) ) ;
#50891=CARTESIAN_POINT ( 'NONE',  ( -111.6028274538085299, -288.7170912920631167, -268.4059816993565164 ) ) ;
#50892=CARTESIAN_POINT ( 'NONE',  ( -87.49538389815894845, -233.3606102865802825, -350.3678815354037965 ) ) ;
#50894=CARTESIAN_POINT ( 'NONE',  ( -110.1264292753925815, -288.7394915632573316, -293.4487458996985083 ) ) ;
#50895=CARTESIAN_POINT ( 'NONE',  ( -93.15992892245486701, -283.5040989628280386, -218.7253317404775430 ) ) ;
#50896=CARTESIAN_POINT ( 'NONE',  ( -56.45459091555333941, -284.7286266506664560, -341.4249788494714721 ) ) ;
#50897=CARTESIAN_POINT ( 'NONE',  ( -87.03102608431292708, -284.5679339385695243, -324.1293253957367142 ) ) ;
#50898=CARTESIAN_POINT ( 'NONE',  ( -67.37466906241759546, -291.4239754838623639, -339.4728216384142456 ) ) ;
#50899=CARTESIAN_POINT ( 'NONE',  ( 22.73918388317162709, -275.2403867254857914, -222.2150498502134610 ) ) ;
#50900=CARTESIAN_POINT ( 'NONE',  ( -83.36943941162631688, -289.5071921624210063, -210.3722277984543894 ) ) ;
#50901=CARTESIAN_POINT ( 'NONE',  ( -45.64961730087578218, -277.1545523770471959, -346.9646729534728706 ) ) ;
#50902=CARTESIAN_POINT ( 'NONE',  ( 20.11494765181627642, -296.1929397740404966, -318.0117258705380436 ) ) ;
#50904=CARTESIAN_POINT ( 'NONE',  ( 31.98288692825981272, -296.4805209788415823, -303.7098442033569654 ) ) ;
#50905=CARTESIAN_POINT ( 'NONE',  ( -1.022770520093521540, -281.2440253241451273, -334.2530488546613014 ) ) ;
#50906=CARTESIAN_POINT ( 'NONE',  ( -112.2152288144974221, -276.6442006766164354, -263.1635230051749090 ) ) ;
#50907=CARTESIAN_POINT ( 'NONE',  ( -110.3678891299274056, -271.3144546575006189, -248.0473400826790851 ) ) ;
#50908=CARTESIAN_POINT ( 'NONE',  ( 9.723352830516123646, -275.7325617673797638, -326.2965580706182323 ) ) ;
#50909=CARTESIAN_POINT ( 'NONE',  ( -63.06066959920939041, -293.2311483973861641, -201.3014165520490053 ) ) ;
#50910=CARTESIAN_POINT ( 'NONE',  ( 2.358014669068211333, -293.5393642680079438, -208.7596732287359771 ) ) ;
#50911=CARTESIAN_POINT ( 'NONE',  ( -33.58661477011126806, -293.5238168183002472, -194.0426691797958370 ) ) ;
#50912=CARTESIAN_POINT ( 'NONE',  ( 26.07468385097006092, -294.2986809761601990, -227.4700500995605807 ) ) ;
#50913=CARTESIAN_POINT ( 'NONE',  ( -63.57097602943072445, -295.2369566199428164, -338.5397463182231377 ) ) ;
#50914=CARTESIAN_POINT ( 'NONE',  ( -17.93200341822250010, -290.8022012981047624, -342.8600548049010968 ) ) ;
#50915=CARTESIAN_POINT ( 'NONE',  ( -102.9169673524919801, -284.1913278749609617, -310.7205571875689998 ) ) ;
#50916=CARTESIAN_POINT ( 'NONE',  ( -80.52658104247448989, -271.6135753591577782, -208.0450735875317037 ) ) ;
#50917=CARTESIAN_POINT ( 'NONE',  ( -3.487441953261195327, -286.3200341203349240, -201.1881542722341862 ) ) ;
#50918=CARTESIAN_POINT ( 'NONE',  ( -67.44334330470294958, -279.4288450031614843, -338.6673247536235749 ) ) ;
#50920=CARTESIAN_POINT ( 'NONE',  ( -85.97784978780988752, -284.1555368381430071, -215.3236148577962297 ) ) ;
#50921=CARTESIAN_POINT ( 'NONE',  ( -29.21975367704297710, -286.9492078422037480, -344.9721863633606063 ) ) ;
#50922=CARTESIAN_POINT ( 'NONE',  ( -70.66955292945459632, -277.7569018184060496, -202.3202500256892051 ) ) ;
#50923=CARTESIAN_POINT ( 'NONE',  ( 116.7412556412048872, 151.1295779098236665, -261.7160256675778101 ) ) ;
#50924=CARTESIAN_POINT ( 'NONE',  ( -70.00431895928686288, -285.1175487550798380, -204.9931896772217215 ) ) ;
#50925=CARTESIAN_POINT ( 'NONE',  ( 35.79203067962625084, -282.4694106255584529, -247.5693182130149239 ) ) ;
#50926=CARTESIAN_POINT ( 'NONE',  ( 12.25465303853404642, -287.4398882375414246, -328.9531137232041260 ) ) ;
#50927=CARTESIAN_POINT ( 'NONE',  ( -97.28681268844545116, -279.5167619965732229, -317.4039059383642893 ) ) ;
#50928=CARTESIAN_POINT ( 'NONE',  ( -84.54884574960647114, -279.0017253002762914, -330.6345996472991260 ) ) ;
#50929=CARTESIAN_POINT ( 'NONE',  ( -95.61046795058176428, -279.0034279764616940, -226.3659374065110796 ) ) ;
#50930=CARTESIAN_POINT ( 'NONE',  ( 20.25220980794826886, -276.8738665047488894, -222.8765063205398747 ) ) ;
#50931=CARTESIAN_POINT ( 'NONE',  ( 39.60688391750915116, -293.5873380482357788, -273.1745524279834854 ) ) ;
#50932=CARTESIAN_POINT ( 'NONE',  ( -83.58454293498222398, -287.7102132997681565, -328.9567346163393040 ) ) ;
#50933=CARTESIAN_POINT ( 'NONE',  ( -1.201436748137719501, -294.1236286711109642, -203.2766802979610645 ) ) ;
#50934=CARTESIAN_POINT ( 'NONE',  ( -73.46665075974691206, -294.4638878973798342, -334.1515092322806595 ) ) ;
#50935=CARTESIAN_POINT ( 'NONE',  ( 35.64259782757726924, -293.1882805918654071, -268.0416916304655501 ) ) ;
#50936=CARTESIAN_POINT ( 'NONE',  ( -110.1418420663086266, -291.9384873975006940, -246.0777937725686968 ) ) ;
#50937=CARTESIAN_POINT ( 'NONE',  ( 32.33099770372923842, -282.4984913336941190, -292.6531239611390447 ) ) ;
#50939=ADVANCED_FACE ( 'NONE', ( #66854 ), #10012, .F. ) ;
#50940=CARTESIAN_POINT ( 'NONE',  ( -81.10637535350065264, -272.5325913237194868, -207.2294969941391685 ) ) ;
#50941=CARTESIAN_POINT ( 'NONE',  ( -73.11907485539609297, -290.1651221641153597, -338.4441452574731670 ) ) ;
#50942=CARTESIAN_POINT ( 'NONE',  ( -27.55550236442894629, -281.0688231859247708, -345.5437479406617740 ) ) ;
#50943=CARTESIAN_POINT ( 'NONE',  ( -37.49728615799227072, -289.3872929793831190, -347.3528851897505660 ) ) ;
#50944=CARTESIAN_POINT ( 'NONE',  ( -44.03053703779866623, -286.2985344710945697, -197.6469725391537793 ) ) ;
#50945=CARTESIAN_POINT ( 'NONE',  ( 24.96937360126054273, -22.70870616253715824, -344.9910381550040483 ) ) ;
#50946=CARTESIAN_POINT ( 'NONE',  ( 159.2431035810776905, 219.8277306504076307, -203.5701272057735878 ) ) ;
#50947=CARTESIAN_POINT ( 'NONE',  ( -93.74409744368286113, -238.7666546281632804, -338.5088866427397534 ) ) ;
#50948=CARTESIAN_POINT ( 'NONE',  ( -105.6614162580993650, -278.0997785501654675, -244.0464234553423069 ) ) ;
#50949=CARTESIAN_POINT ( 'NONE',  ( -87.73316560708165923, -278.2487418301028015, -217.0469511595870244 ) ) ;
#50950=CARTESIAN_POINT ( 'NONE',  ( -3.831473428062826425, -274.1488981792788309, -201.0443114855024476 ) ) ;
#50951=CARTESIAN_POINT ( 'NONE',  ( -110.4560631405595643, -273.2888399267177419, -270.3704977824100979 ) ) ;
#50952=CARTESIAN_POINT ( 'NONE',  ( -113.4552190830244456, -277.2189962577540996, -263.0520944849046714 ) ) ;
#50953=CARTESIAN_POINT ( 'NONE',  ( -88.06460109016667559, -281.7856572128818584, -325.1952930489084110 ) ) ;
#50954=CARTESIAN_POINT ( 'NONE',  ( -74.09630248089541737, -297.2933515904690012, -336.9262263504716657 ) ) ;
#50955=CARTESIAN_POINT ( 'NONE',  ( -32.15917367351151768, -292.6116002623460872, -197.4709880223978473 ) ) ;
#50956=CARTESIAN_POINT ( 'NONE',  ( -99.26624624139137154, -288.6931917087532611, -309.9413411553215951 ) ) ;
#50957=CARTESIAN_POINT ( 'NONE',  ( -3.877972876050205908, -275.1334331069022028, -201.1115825374340886 ) ) ;
#50958=CARTESIAN_POINT ( 'NONE',  ( -97.18216028420732755, -296.1358376802232897, -312.1716349946260038 ) ) ;
#50962=CARTESIAN_POINT ( 'NONE',  ( -92.04838421226122591, -281.1990888989095083, -218.1663481207656616 ) ) ;
#50963=CARTESIAN_POINT ( 'NONE',  ( -46.50868548182884155, -281.0128985697700159, -197.5760893315352575 ) ) ;
#50964=CARTESIAN_POINT ( 'NONE',  ( -9.256757258909233954, -282.1744649884686851, -199.7550984223298940 ) ) ;
#50965=CARTESIAN_POINT ( 'NONE',  ( -10.90197354023956677, -281.7576543484078115, -338.7109086237585416 ) ) ;
#50966=CARTESIAN_POINT ( 'NONE',  ( -68.55882751477295756, -272.1142347183406400, -203.5925259070333766 ) ) ;
#50969=CARTESIAN_POINT ( 'NONE',  ( 36.42793918752401794, -276.0826956006137038, -248.6764523678102421 ) ) ;
#50971=CARTESIAN_POINT ( 'NONE',  ( 20.21266117828161057, -278.2166602070761883, -318.4495380733854972 ) ) ;
#50972=CARTESIAN_POINT ( 'NONE',  ( -12.07825596151696956, -275.3045789554300313, -342.5301652189041874 ) ) ;
#50975=CARTESIAN_POINT ( 'NONE',  ( -75.89425137132091947, -285.5437228061603037, -335.1680927717017084 ) ) ;
#50976=CARTESIAN_POINT ( 'NONE',  ( 29.63378567290673971, -293.1445530632305463, -299.8040463046418154 ) ) ;
#50977=CARTESIAN_POINT ( 'NONE',  ( -33.72381460238398176, -285.4451497863647091, -193.5482044125795937 ) ) ;
#50978=CARTESIAN_POINT ( 'NONE',  ( -95.93217628199963087, -282.1638250617883159, -315.6049286642285097 ) ) ;
#50979=CARTESIAN_POINT ( 'NONE',  ( -10.77989302364126800, -281.2737121324661302, -339.0434373999217428 ) ) ;
#50980=CARTESIAN_POINT ( 'NONE',  ( 12.19592657620327891, -283.5492645987591800, -324.5197188179855061 ) ) ;
#50981=CARTESIAN_POINT ( 'NONE',  ( -66.72791628044898005, -271.6670035016841780, -201.3578502986385388 ) ) ;
#50982=CARTESIAN_POINT ( 'NONE',  ( -111.1057353475587917, -282.7097134914578191, -289.5259226527679743 ) ) ;
#50983=CARTESIAN_POINT ( 'NONE',  ( -109.2893851079527252, -298.2790390368232352, -291.5849199021723734 ) ) ;
#50984=CARTESIAN_POINT ( 'NONE',  ( -91.47880715477889169, -280.1983502611237782, -221.0399045835715697 ) ) ;
#50985=CARTESIAN_POINT ( 'NONE',  ( -51.84510091347816285, -287.8672905728646469, -196.5538343999191113 ) ) ;
#50988=CARTESIAN_POINT ( 'NONE',  ( 34.90286814260568349, -295.1890382577763035, -248.2243487094521015 ) ) ;
#50989=CARTESIAN_POINT ( 'NONE',  ( -48.94163486376639582, -275.1996230818745630, -344.5114353270543575 ) ) ;
#50990=CARTESIAN_POINT ( 'NONE',  ( -41.76150947437994176, -288.3036439178633259, -347.0856160532400736 ) ) ;
#50991=CARTESIAN_POINT ( 'NONE',  ( 25.54008364571286549, -291.4241584403899878, -231.6334817727388895 ) ) ;
#50992=CARTESIAN_POINT ( 'NONE',  ( -40.54390445751135275, -275.7780482727015396, -343.7970234432891061 ) ) ;
#50993=CARTESIAN_POINT ( 'NONE',  ( -91.32142545007197043, -293.9692792276212003, -321.3964809502224966 ) ) ;
#50994=CARTESIAN_POINT ( 'NONE',  ( -105.1645984978421069, -292.2460609290928915, -241.9214067118645914 ) ) ;
#50995=CARTESIAN_POINT ( 'NONE',  ( -20.19161114001083490, -285.3376638359844719, -345.3538533559490702 ) ) ;
#50996=CARTESIAN_POINT ( 'NONE',  ( 23.46465375207146309, -292.6518335754161058, -316.4620407769572239 ) ) ;
#50997=CARTESIAN_POINT ( 'NONE',  ( -18.24707915307216410, -290.4022335897068956, -341.7012804433098268 ) ) ;
#50998=CARTESIAN_POINT ( 'NONE',  ( -113.1751167339738089, -288.8531414278379543, -265.5375365763666196 ) ) ;
#51000=CARTESIAN_POINT ( 'NONE',  ( 31.03938911176018678, -289.3399650551003788, -297.6905788816848144 ) ) ;
#51001=CARTESIAN_POINT ( 'NONE',  ( -101.7805382291104195, -290.8823059450201640, -305.1129508036477205 ) ) ;
#51003=CARTESIAN_POINT ( 'NONE',  ( -72.97547648096811201, -290.7186951878180707, -338.1861407105386661 ) ) ;
#51004=CARTESIAN_POINT ( 'NONE',  ( -95.53087620390357415, -277.2296967769691491, -222.4617682166225165 ) ) ;
#51005=CARTESIAN_POINT ( 'NONE',  ( -22.57439544081095661, -280.5693661488294879, -194.7577481575451941 ) ) ;
#51006=CARTESIAN_POINT ( 'NONE',  ( 39.16225703207692277, -281.1062278192027293, -261.3566547280000805 ) ) ;
#51007=CARTESIAN_POINT ( 'NONE',  ( 29.45056055819301477, -285.0995438406746416, -236.1321022833115251 ) ) ;
#51009=CARTESIAN_POINT ( 'NONE',  ( 31.47078313542831651, -280.0585113518169464, -298.2126462205336566 ) ) ;
#51010=CARTESIAN_POINT ( 'NONE',  ( -75.07780795924897177, -283.5496724866497402, -205.4863033057050927 ) ) ;
#51012=CARTESIAN_POINT ( 'NONE',  ( -94.70250776891384703, -276.3448881708775389, -320.6845270535447412 ) ) ;
#51013=CARTESIAN_POINT ( 'NONE',  ( -110.8157998883666266, -283.1950498810738281, -292.3851274451994300 ) ) ;
#51014=CARTESIAN_POINT ( 'NONE',  ( -110.0473752105498164, -273.4623154001432681, -262.2071902407515154 ) ) ;
#51015=CARTESIAN_POINT ( 'NONE',  ( -69.38316837066221865, -293.2235294107999266, -203.8657005363225494 ) ) ;
#51016=CARTESIAN_POINT ( 'NONE',  ( -111.2530440437265469, -274.2242566822889103, -250.7749510710396521 ) ) ;
#51017=CARTESIAN_POINT ( 'NONE',  ( 35.71992156475009494, -275.2350692071352114, -271.5895561323770835 ) ) ;
#51018=CARTESIAN_POINT ( 'NONE',  ( -91.84357065002804177, -297.8292329132049190, -321.9581749194084068 ) ) ;
#51019=CARTESIAN_POINT ( 'NONE',  ( -80.53885857708523588, -289.7865310167421171, -334.1672384920702257 ) ) ;
#51020=CARTESIAN_POINT ( 'NONE',  ( 25.10460180199353886, -279.0592042294516091, -227.7283495288590132 ) ) ;
#51021=CARTESIAN_POINT ( 'NONE',  ( -3.319439481211793996, -292.3223121054058424, -201.2706379079105545 ) ) ;
#51022=CARTESIAN_POINT ( 'NONE',  ( -44.31070046219010550, -291.0207325948613857, -197.4071773135576677 ) ) ;
#51023=CARTESIAN_POINT ( 'NONE',  ( 21.58408446128172642, -292.1892730909928559, -316.7794793842076047 ) ) ;
#51026=CARTESIAN_POINT ( 'NONE',  ( -110.1845341748307874, -289.9771885154749498, -276.6289519616127563 ) ) ;
#51028=CARTESIAN_POINT ( 'NONE',  ( -37.99251322539671349, -286.9854318925292773, -193.5991700109078408 ) ) ;
#51029=CARTESIAN_POINT ( 'NONE',  ( -92.05005921254146983, -286.4090924074130839, -314.0302885647153062 ) ) ;
#51030=CARTESIAN_POINT ( 'NONE',  ( -11.14879584051634076, -293.7778559617395331, -342.5753377799391615 ) ) ;
#51031=CARTESIAN_POINT ( 'NONE',  ( 38.78916494465794784, -282.9691339289838083, -278.4496375185593706 ) ) ;
#51032=CARTESIAN_POINT ( 'NONE',  ( -96.57358185941994577, -284.9823984878326542, -227.6714896863678916 ) ) ;
#51033=CARTESIAN_POINT ( 'NONE',  ( -1.112648095701359141, -278.0826014965762170, -334.5917887401917596 ) ) ;
#51034=CARTESIAN_POINT ( 'NONE',  ( -50.79178153345812774, -293.2449305763212237, -343.7841532648337761 ) ) ;
#51035=CARTESIAN_POINT ( 'NONE',  ( 22.15422249566766766, -295.9210824752074132, -314.3862154445993156 ) ) ;
#51036=CARTESIAN_POINT ( 'NONE',  ( 34.55041386389184055, -274.5410830132706224, -285.1480869662650548 ) ) ;
#51039=CARTESIAN_POINT ( 'NONE',  ( -24.91541006873382713, -294.5646587161193679, -346.3844490381481478 ) ) ;
#51040=CARTESIAN_POINT ( 'NONE',  ( -28.98771047613502461, -290.8655955160263602, -344.3308756797667343 ) ) ;
#51041=CARTESIAN_POINT ( 'NONE',  ( -81.68173343236078665, -296.7195798862911715, -332.9995598328504229 ) ) ;
#51042=CARTESIAN_POINT ( 'NONE',  ( -38.63501986142806288, -286.6869602755991764, -197.2581271832783898 ) ) ;
#51043=CARTESIAN_POINT ( 'NONE',  ( -95.04187543518484915, -276.9236646183248354, -320.9922347279758696 ) ) ;
#51044=CARTESIAN_POINT ( 'NONE',  ( -61.55159473342654763, -296.0098837190847689, -343.4044083551847848 ) ) ;
#51045=CARTESIAN_POINT ( 'NONE',  ( -29.13490488666295164, -287.0889298664189369, -345.7327989286015963 ) ) ;
#51046=CARTESIAN_POINT ( 'NONE',  ( -111.1939019949068239, -296.6124288744349542, -292.1238771964989951 ) ) ;
#51047=CARTESIAN_POINT ( 'NONE',  ( -65.33899087563729324, -292.0091314203624506, -202.9069649173861194 ) ) ;
#51050=CARTESIAN_POINT ( 'NONE',  ( 202.8072765148675103, 291.9636416985566143, -68.23872395582101547 ) ) ;
#51051=CARTESIAN_POINT ( 'NONE',  ( -40.80456282695320169, -287.5295882308791988, -194.0813409114329602 ) ) ;
#51052=CARTESIAN_POINT ( 'NONE',  ( -55.56934967048407970, -283.3380690714490697, -190.3538533559490702 ) ) ;
#51054=CARTESIAN_POINT ( 'NONE',  ( -104.7003003547445417, -278.3818676540418551, -233.2648680129257457 ) ) ;
#51055=CARTESIAN_POINT ( 'NONE',  ( -88.15549523683108646, -285.7650690500026940, -325.3681939281526638 ) ) ;
#51056=CARTESIAN_POINT ( 'NONE',  ( -108.7587668370613301, -282.7786464165852180, -297.6786500538951259 ) ) ;
#51057=CARTESIAN_POINT ( 'NONE',  ( -56.45853184964177984, -287.3801278799319903, -342.3581729291028068 ) ) ;
#51058=CARTESIAN_POINT ( 'NONE',  ( 11.91976159537290769, -278.2363651558653146, -327.9251159915700100 ) ) ;
#51059=CARTESIAN_POINT ( 'NONE',  ( -35.15172674704856348, -298.5726437816636576, -197.2993898346907429 ) ) ;
#51060=EDGE_CURVE ( 'NONE', #92061, #92001, #3796, .T. ) ;
#51061=CARTESIAN_POINT ( 'NONE',  ( -63.76181381131007697, -294.0886479231024282, -338.9950778410869816 ) ) ;
#51062=CARTESIAN_POINT ( 'NONE',  ( 6.119804185979267785, -281.2766240399240019, -206.9228769201384353 ) ) ;
#51063=CARTESIAN_POINT ( 'NONE',  ( -36.46617441205170707, -277.0409132872975988, -343.3683347522843405 ) ) ;
#51064=CARTESIAN_POINT ( 'NONE',  ( -108.3867763994746127, -278.1276044459845025, -253.1422386305939369 ) ) ;
#51065=CARTESIAN_POINT ( 'NONE',  ( 36.98224627476096060, -276.3942870809443093, -251.4549416924350851 ) ) ;
#51066=CARTESIAN_POINT ( 'NONE',  ( -11.98142676218160574, -275.6501241513911964, -342.7932557989564089 ) ) ;
#51067=CARTESIAN_POINT ( 'NONE',  ( -71.48678950961217993, -195.9896530788094253, -360.3036401658151817 ) ) ;
#51068=CARTESIAN_POINT ( 'NONE',  ( -77.13658905977014513, -275.5849227701816062, -333.9932805167524634 ) ) ;
#51070=CARTESIAN_POINT ( 'NONE',  ( -112.6201739033270997, -297.8084888185636601, -283.7653447835110114 ) ) ;
#51073=CARTESIAN_POINT ( 'NONE',  ( -42.71042936018697134, -287.0625339764642376, -197.2361771341240910 ) ) ;
#51074=CARTESIAN_POINT ( 'NONE',  ( -15.72349531265234823, -288.0880960616462403, -197.4598595427160035 ) ) ;
#51075=CARTESIAN_POINT ( 'NONE',  ( -49.43022779396378041, -285.2426830650466627, -198.2140551011335674 ) ) ;
#51076=CARTESIAN_POINT ( 'NONE',  ( -83.92712333052770646, -277.8001142140955722, -213.0565520483397961 ) ) ;
#51077=CARTESIAN_POINT ( 'NONE',  ( -108.5463921900058892, -286.6878300636243466, -249.1884143319376221 ) ) ;
#51078=CARTESIAN_POINT ( 'NONE',  ( -109.5628939842647327, -277.2243763405871846, -255.6415385081728857 ) ) ;
#51079=CARTESIAN_POINT ( 'NONE',  ( -21.53071167818425735, -278.1604891875282419, -342.1857161561738394 ) ) ;
#51080=CARTESIAN_POINT ( 'NONE',  ( 31.17385357820676006, -275.7064907657397157, -244.9917005299174946 ) ) ;
#51081=CARTESIAN_POINT ( 'NONE',  ( 36.39799149660461097, -286.6089816499899143, -291.1568765219308261 ) ) ;
#51082=CARTESIAN_POINT ( 'NONE',  ( 39.54879918530137672, -282.3494671859059508, -269.9209668513495330 ) ) ;
#51083=CARTESIAN_POINT ( 'NONE',  ( 38.60810804908933846, -282.1994100333202482, -282.7379071919000353 ) ) ;
#51086=FACE_BOUND ( 'NONE', #20335, .T. ) ;
#51087=CARTESIAN_POINT ( 'NONE',  ( 20.56060653380401604, -290.0815428073241833, -319.2244822390707668 ) ) ;
#51088=CARTESIAN_POINT ( 'NONE',  ( -74.20449915820179854, -288.2163608899847986, -337.4166041082575589 ) ) ;
#51089=CARTESIAN_POINT ( 'NONE',  ( -16.70375795726870294, -296.3901479883312504, -343.7677806324035714 ) ) ;
#51090=CARTESIAN_POINT ( 'NONE',  ( 51.92734036832234779, -298.3949240948066972, -197.2122406934001617 ) ) ;
#51091=CARTESIAN_POINT ( 'NONE',  ( -56.15580824353236267, -291.1646794034347181, -195.7452483575337112 ) ) ;
#51092=CARTESIAN_POINT ( 'NONE',  ( 28.28430794893779776, -285.5795050992591655, -236.7234117582345334 ) ) ;
#51093=CARTESIAN_POINT ( 'NONE',  ( -47.10627101322353383, -290.1662694622758067, -196.9947280787739601 ) ) ;
#51095=CARTESIAN_POINT ( 'NONE',  ( 14.37398244000208081, -289.5099409172001970, -322.4439239837490732 ) ) ;
#51096=CARTESIAN_POINT ( 'NONE',  ( -69.91165696735023971, -300.1233781216987495, -202.8022627189028810 ) ) ;
#51097=CARTESIAN_POINT ( 'NONE',  ( -18.20929502808394673, -290.8057285049814027, -342.8797481467224202 ) ) ;
#51098=CARTESIAN_POINT ( 'NONE',  ( -5.142081507021530662, -286.6291991882284265, -338.2958874063808139 ) ) ;
#51099=CARTESIAN_POINT ( 'NONE',  ( -98.31313142189650023, -291.9579171654473839, -314.0576789665474280 ) ) ;
#51100=CARTESIAN_POINT ( 'NONE',  ( -107.6143234067178440, -285.2209477664488304, -291.0254421079523581 ) ) ;
#51101=CARTESIAN_POINT ( 'NONE',  ( -55.76469888281305032, -293.8158264128625774, -197.4334616761163375 ) ) ;
#51103=APPLICATION_CONTEXT ( 'automotive_design' ) ;
#51105=CARTESIAN_POINT ( 'NONE',  ( -110.2338880845598936, -274.7787865676199885, -251.0526395367190844 ) ) ;
#51106=CARTESIAN_POINT ( 'NONE',  ( 33.80478422507519554, -280.9744704911740882, -287.4666434848887775 ) ) ;
#51107=CARTESIAN_POINT ( 'NONE',  ( -38.95290268266872147, -281.0721757505338019, -345.3566466280354916 ) ) ;
#51108=CARTESIAN_POINT ( 'NONE',  ( -84.09507087535742187, -294.8732843839204065, -331.4059196420202511 ) ) ;
#51109=CARTESIAN_POINT ( 'NONE',  ( 32.07639937149461673, -273.4543652466414869, -244.6881463194227422 ) ) ;
#51110=CARTESIAN_POINT ( 'NONE',  ( -57.00361218945658237, -275.3874260833529775, -342.2110595009923486 ) ) ;
#51111=CARTESIAN_POINT ( 'NONE',  ( -110.8773036433820920, -297.8525773782296255, -271.4872749191334833 ) ) ;
#51113=CARTESIAN_POINT ( 'NONE',  ( -99.19686102394565808, -294.1986119463037426, -314.5849452550909859 ) ) ;
#51114=CARTESIAN_POINT ( 'NONE',  ( 1.899267874983875171, -295.9415172121264277, -332.6751630027971487 ) ) ;
#51116=CARTESIAN_POINT ( 'NONE',  ( -28.86714660428147283, -295.7449464245688091, -343.0812458012580350 ) ) ;
#51118=CARTESIAN_POINT ( 'NONE',  ( -109.1265359876504704, -282.2773268986495623, -293.3241030871791963 ) ) ;
#51119=CARTESIAN_POINT ( 'NONE',  ( -92.74440614636914404, -297.2290146111806166, -222.8072700936497483 ) ) ;
#51120=CARTESIAN_POINT ( 'NONE',  ( -102.9180786539602792, -284.0246746958243875, -310.7187514541928408 ) ) ;
#51121=CARTESIAN_POINT ( 'NONE',  ( 24.76100957757790511, -284.0519538684512213, -313.4253478896217757 ) ) ;
#51123=CARTESIAN_POINT ( 'NONE',  ( 22.38604925080206343, -287.8707831529797545, -318.9446070580681862 ) ) ;
#51124=CARTESIAN_POINT ( 'NONE',  ( -2.767129051994785538, -290.5102143224892188, -203.9937505166963376 ) ) ;
#51126=CARTESIAN_POINT ( 'NONE',  ( -111.5723750715653324, -277.9989432986553766, -250.4617769120534092 ) ) ;
#51128=CARTESIAN_POINT ( 'NONE',  ( 35.78497577281001440, -278.8380690714489560, -253.7030783399848985 ) ) ;
#51130=CARTESIAN_POINT ( 'NONE',  ( 34.96124105455808717, -286.1776501377624413, -257.4481184333653800 ) ) ;
#51131=CARTESIAN_POINT ( 'NONE',  ( -104.8902311795035445, -289.0011005629708052, -306.6748682947091993 ) ) ;
#51134=CARTESIAN_POINT ( 'NONE',  ( -97.54704456335279872, -298.7417860848294140, -227.6790735431856945 ) ) ;
#51135=CARTESIAN_POINT ( 'NONE',  ( -112.4828521586852048, -279.8016968538092897, -284.3042359674442423 ) ) ;
#51136=CARTESIAN_POINT ( 'NONE',  ( -96.04872799750523882, -295.2192699766738428, -223.1182170727707899 ) ) ;
#51137=CARTESIAN_POINT ( 'NONE',  ( 32.75607713922430975, -280.9483591675636944, -249.9065559243356631 ) ) ;
#51138=CARTESIAN_POINT ( 'NONE',  ( 6.615742610128464207, -294.6396333603258313, -333.6458882556190702 ) ) ;
#51139=CARTESIAN_POINT ( 'NONE',  ( 22.73174121994457408, -285.0091164189876736, -224.5087289828665291 ) ) ;
#51140=CARTESIAN_POINT ( 'NONE',  ( -111.3220646130688323, -280.3940606587116804, -282.6861462060236363 ) ) ;
#51141=CARTESIAN_POINT ( 'NONE',  ( -75.32245294360193100, -296.5914191786604306, -207.6854697250635979 ) ) ;
#51143=CARTESIAN_POINT ( 'NONE',  ( 18.85951277953860128, -284.2174640594336097, -319.4861673201651229 ) ) ;
#51145=CARTESIAN_POINT ( 'NONE',  ( 21.31550574532286291, -290.4094976428776249, -223.6242672951989618 ) ) ;
#51146=CARTESIAN_POINT ( 'NONE',  ( 4.783199877688997681, -273.8022978453109317, -206.0356185755451293 ) ) ;
#51147=CARTESIAN_POINT ( 'NONE',  ( -104.0485805477667043, -289.9848100426735868, -300.1371361625018608 ) ) ;
#51148=CARTESIAN_POINT ( 'NONE',  ( 3.068151096329007732, -282.1253954055514441, -208.6739960586112090 ) ) ;
#51149=CARTESIAN_POINT ( 'NONE',  ( -46.29582928246363593, -275.5367938077609438, -197.1063298430928228 ) ) ;
#51150=CARTESIAN_POINT ( 'NONE',  ( 0.4890743226171061497, -284.1569440888880536, -336.5220397580550298 ) ) ;
#51151=CARTESIAN_POINT ( 'NONE',  ( 19.99577512790231637, -279.7032604210278919, -224.5403318966637869 ) ) ;
#51152=CARTESIAN_POINT ( 'NONE',  ( -108.1440564277788496, -280.2301735133773377, -295.2576465013926281 ) ) ;
#51153=CARTESIAN_POINT ( 'NONE',  ( -97.81438414798213898, -273.3563534167021203, -222.6950452267130345 ) ) ;
#51154=CARTESIAN_POINT ( 'NONE',  ( -41.19064645770409072, -273.8384209096070663, -193.4051156341953401 ) ) ;
#51155=CARTESIAN_POINT ( 'NONE',  ( 28.44185374688795420, -295.9390054384124937, -305.3115145383727622 ) ) ;
#51157=CARTESIAN_POINT ( 'NONE',  ( -16.86387529450534828, -292.9301606725258580, -343.3603985373750334 ) ) ;
#51158=CARTESIAN_POINT ( 'NONE',  ( -24.57952629240084264, -273.7269398815510044, -198.3712105745552492 ) ) ;
#51159=CARTESIAN_POINT ( 'NONE',  ( 12.80811989866018230, -294.2574092503788847, -212.8484819595923909 ) ) ;
#51160=CARTESIAN_POINT ( 'NONE',  ( 31.95455697924148097, -283.6233781216988064, -236.9535640164627637 ) ) ;
#51161=CARTESIAN_POINT ( 'NONE',  ( -66.87660097890348254, -292.8786753979895252, -199.6808636619570052 ) ) ;
#51162=CARTESIAN_POINT ( 'NONE',  ( -85.85465383972889697, -291.7255569108441478, -327.4077514720813156 ) ) ;
#51163=CARTESIAN_POINT ( 'NONE',  ( -18.58133240007699882, -274.8097791813563049, -342.8047307183484236 ) ) ;
#51164=CARTESIAN_POINT ( 'NONE',  ( -15.94400305952446395, -278.6935536367594750, -341.7135144517626486 ) ) ;
#51165=CARTESIAN_POINT ( 'NONE',  ( -7.431721254557253964, -292.7367500436675414, -338.5417221535161616 ) ) ;
#51166=CARTESIAN_POINT ( 'NONE',  ( 37.21439624702472315, -283.5848084734714121, -283.9126926997171836 ) ) ;
#51168=CARTESIAN_POINT ( 'NONE',  ( -90.75982214474217358, -283.5031429853315217, -320.1465749655091031 ) ) ;
#51169=CARTESIAN_POINT ( 'NONE',  ( 20.82264648940808627, -281.9542099770382606, -220.3571436467458682 ) ) ;
#51170=CARTESIAN_POINT ( 'NONE',  ( 21.29611585587976919, -281.0142438009466446, -319.6522455459171965 ) ) ;
#51171=CARTESIAN_POINT ( 'NONE',  ( -6.657707155575216973, -277.6003056939377416, -340.7408971148583419 ) ) ;
#51173=CARTESIAN_POINT ( 'NONE',  ( 35.40752252100414665, -277.3643215082681195, -293.3884573108048244 ) ) ;
#51174=CARTESIAN_POINT ( 'NONE',  ( -37.30987171927208124, -291.5519495502701375, -340.3611179825599606 ) ) ;
#51176=CARTESIAN_POINT ( 'NONE',  ( -97.72529541505058148, -299.1593410108936268, -225.8554737236963206 ) ) ;
#51177=CARTESIAN_POINT ( 'NONE',  ( -46.12613884528399666, -275.1840826853351132, -344.5389969121603144 ) ) ;
#51178=CARTESIAN_POINT ( 'NONE',  ( -112.1779767200939233, -292.4792220396324751, -257.1889609516422297 ) ) ;
#51179=CARTESIAN_POINT ( 'NONE',  ( 35.39763592381030577, -292.7984871376878004, -262.5993243562664361 ) ) ;
#51180=CARTESIAN_POINT ( 'NONE',  ( -4.365129471991358479, -288.1367683650125286, -339.8886968637668815 ) ) ;
#51182=CARTESIAN_POINT ( 'NONE',  ( 10.81279845429053843, -292.9762589657690910, -329.7567760583565359 ) ) ;
#51183=CARTESIAN_POINT ( 'NONE',  ( -78.84315096917276833, -282.0217828831396218, -331.3862766615405917 ) ) ;
#51184=CARTESIAN_POINT ( 'NONE',  ( -45.47463465081332856, -291.0167197691744150, -344.1494697427020242 ) ) ;
#51185=CARTESIAN_POINT ( 'NONE',  ( -90.14627724528926933, -283.7690935259753360, -218.8837821325069797 ) ) ;
#51186=CARTESIAN_POINT ( 'NONE',  ( -66.74157205310883967, -284.7607549507834506, -337.7312264360124345 ) ) ;
#51187=CARTESIAN_POINT ( 'NONE',  ( -26.16693419948606092, -289.8544500578014436, -346.3081048805617002 ) ) ;
#51188=CARTESIAN_POINT ( 'NONE',  ( 25.18570854657578550, -281.5235480821974647, -232.4700798614151722 ) ) ;
#51189=CARTESIAN_POINT ( 'NONE',  ( -22.19116521235297057, -293.6571598072058578, -345.4508643481782997 ) ) ;
#51190=CARTESIAN_POINT ( 'NONE',  ( -31.82813607470581019, -289.7872086811860299, -347.0540191270774244 ) ) ;
#51191=CARTESIAN_POINT ( 'NONE',  ( 39.29276794509681281, -287.9518246092063691, -262.9569427667189530 ) ) ;
#51192=CARTESIAN_POINT ( 'NONE',  ( -87.69603675152850997, -285.4913477055930002, -217.5081068317804238 ) ) ;
#51195=CARTESIAN_POINT ( 'NONE',  ( 25.50067708387251031, -295.9792269590741398, -312.6829930222918961 ) ) ;
#51196=CARTESIAN_POINT ( 'NONE',  ( -109.8834738408593239, -294.9288911563629085, -294.6713902756424659 ) ) ;
#51197=CARTESIAN_POINT ( 'NONE',  ( -96.28950371176620138, -277.0035426759324082, -313.8397643539821615 ) ) ;
#51198=CARTESIAN_POINT ( 'NONE',  ( 53.44637165907408871, -298.5094331931565534, -193.4727354929377441 ) ) ;
#51199=CARTESIAN_POINT ( 'NONE',  ( -71.26705041534634688, -293.9883632973611043, -335.7952516704156665 ) ) ;
#51200=CARTESIAN_POINT ( 'NONE',  ( -13.76355686666970080, -276.1225486433998526, -200.2038291762643212 ) ) ;
#51201=CARTESIAN_POINT ( 'NONE',  ( -106.7483883185292370, -295.1318010299526122, -244.5096044230448058 ) ) ;
#51202=CARTESIAN_POINT ( 'NONE',  ( 23.26952443796387371, -295.3311244716243777, -311.8433769586935114 ) ) ;
#51203=CARTESIAN_POINT ( 'NONE',  ( 34.78483564400909955, -294.4586391219061738, -257.1769313256421583 ) ) ;
#51205=CARTESIAN_POINT ( 'NONE',  ( -109.4636967734172259, -294.2793639751031378, -291.5831153897665331 ) ) ;
#51206=CARTESIAN_POINT ( 'NONE',  ( -97.91123680697840825, -275.1561204526838651, -226.0443558784494655 ) ) ;
#51207=CARTESIAN_POINT ( 'NONE',  ( -34.55708599290608163, -289.9577002517169149, -343.5931953528137797 ) ) ;
#51208=CARTESIAN_POINT ( 'NONE',  ( -70.93675025342905371, -295.8414667259179396, -335.2092027438978334 ) ) ;
#51209=CARTESIAN_POINT ( 'NONE',  ( -100.5261445489632024, -281.0841476157992247, -229.2041049313961594 ) ) ;
#51210=CARTESIAN_POINT ( 'NONE',  ( -50.83609103335521695, -278.5680249251117289, -195.0537499125560430 ) ) ;
#51211=CARTESIAN_POINT ( 'NONE',  ( 24.28099457999335087, -275.5134893412964061, -316.3606428042467655 ) ) ;
#51212=CARTESIAN_POINT ( 'NONE',  ( -69.65595943882617291, -281.5607536458534241, -337.4356376623857727 ) ) ;
#51213=CARTESIAN_POINT ( 'NONE',  ( -38.14086047152152759, -278.4421721935345317, -194.1653060168162028 ) ) ;
#51214=CARTESIAN_POINT ( 'NONE',  ( -72.87592414889944337, -277.5824163051257187, -204.1094712698206592 ) ) ;
#51215=CARTESIAN_POINT ( 'NONE',  ( 9.338798127652633951, -297.3333334804277115, -196.8786743985532439 ) ) ;
#51216=CARTESIAN_POINT ( 'NONE',  ( -25.29944381291146982, -276.2056926635384571, -196.2821725839788769 ) ) ;
#51219=CARTESIAN_POINT ( 'NONE',  ( -95.14593035939897447, -287.9073109253796474, -318.7244731886689237 ) ) ;
#51220=CARTESIAN_POINT ( 'NONE',  ( -113.3600532252344095, -290.3988737420636994, -282.6171366018573963 ) ) ;
#51221=CARTESIAN_POINT ( 'NONE',  ( 32.99699653898910867, -277.2087980014251229, -243.8564735617798078 ) ) ;
#51222=CARTESIAN_POINT ( 'NONE',  ( -78.49956315542313234, -295.4969896288704376, -207.8003928352211176 ) ) ;
#51224=CARTESIAN_POINT ( 'NONE',  ( -78.42747205029628788, -284.7112635484882617, -205.4294757285993853 ) ) ;
#51227=CARTESIAN_POINT ( 'NONE',  ( -65.70949196615140409, -283.6811203973288116, -200.8785762500826877 ) ) ;
#51229=CARTESIAN_POINT ( 'NONE',  ( 35.93213221121447987, -292.2807214703314571, -265.3041903316326398 ) ) ;
#51230=CARTESIAN_POINT ( 'NONE',  ( -88.52937113728961549, -283.4645782699816436, -216.5960008964246981 ) ) ;
#51233=CARTESIAN_POINT ( 'NONE',  ( 36.28297239206418823, -291.7355669292099378, -284.6582592317561762 ) ) ;
#51234=CARTESIAN_POINT ( 'NONE',  ( -78.79941748305679994, -282.0798711219177903, -334.4233176276492259 ) ) ;
#51235=CARTESIAN_POINT ( 'NONE',  ( -110.0710376239063066, -279.9878725310821892, -282.9610248752762232 ) ) ;
#51236=CARTESIAN_POINT ( 'NONE',  ( -113.9437735332358415, -285.7617775967707985, -269.9990855383693429 ) ) ;
#51237=CARTESIAN_POINT ( 'NONE',  ( -73.55563123900545008, -285.5572424245465868, -206.9624662142850298 ) ) ;
#51238=CARTESIAN_POINT ( 'NONE',  ( -91.38836361919092610, -279.2651496445404291, -320.3785164674092698 ) ) ;
#51239=CARTESIAN_POINT ( 'NONE',  ( -110.3204390218664770, -279.4230098878219906, -265.1933915910096289 ) ) ;
#51240=CARTESIAN_POINT ( 'NONE',  ( -111.5135156720319429, -286.6994352803285437, -258.9029224791194110 ) ) ;
#51243=CARTESIAN_POINT ( 'NONE',  ( -113.9434354656293777, -296.2876553284954184, -278.1825083814383106 ) ) ;
#51244=CARTESIAN_POINT ( 'NONE',  ( 6.837977664251367216, -290.4280544449424610, -330.5920098815333859 ) ) ;
#51246=CARTESIAN_POINT ( 'NONE',  ( -72.08107566293803359, -282.1233781216987495, -198.2974183793908196 ) ) ;
#51247=CARTESIAN_POINT ( 'NONE',  ( -61.93543364288468922, -278.6602465554441324, -197.6646250129299744 ) ) ;
#51248=CARTESIAN_POINT ( 'NONE',  ( 31.47236698863065740, -291.5267467177152980, -237.5113012651123654 ) ) ;
#51249=CARTESIAN_POINT ( 'NONE',  ( 13.60503044792356775, -288.3012470983588287, -217.0447169430276517 ) ) ;
#51250=CARTESIAN_POINT ( 'NONE',  ( -111.2916997068601574, -280.2724700465123533, -273.4224205519616930 ) ) ;
#51251=CARTESIAN_POINT ( 'NONE',  ( 35.82646053970353250, -289.2564825129219912, -292.4299170415991398 ) ) ;
#51252=CARTESIAN_POINT ( 'NONE',  ( -104.8007342804427253, -286.1190163130639803, -303.2565073990449491 ) ) ;
#51253=CARTESIAN_POINT ( 'NONE',  ( -112.7932035111290219, -278.5258611049355295, -285.7908604842945692 ) ) ;
#51254=CARTESIAN_POINT ( 'NONE',  ( -37.11996792456957195, -296.0750594714473891, -195.7134715578960709 ) ) ;
#51255=CARTESIAN_POINT ( 'NONE',  ( 38.27064004391357344, -291.6316672520829343, -270.3353211111757446 ) ) ;
#51256=CARTESIAN_POINT ( 'NONE',  ( -77.49070475511013001, -279.3628606267507166, -204.5950748890428770 ) ) ;
#51257=CARTESIAN_POINT ( 'NONE',  ( -31.26177024751022770, -275.9901474282495997, -196.3624454328090678 ) ) ;
#51259=CARTESIAN_POINT ( 'NONE',  ( 31.98288692825981272, -296.4805209788415823, -303.7098442033569654 ) ) ;
#51260=CARTESIAN_POINT ( 'NONE',  ( 15.34083055876097212, -273.0241809487641262, -215.6023289834772640 ) ) ;
#51262=CARTESIAN_POINT ( 'NONE',  ( -103.4228329088073082, -278.4819740116267894, -239.0769838463497479 ) ) ;
#51263=CARTESIAN_POINT ( 'NONE',  ( -20.19995125228745536, -278.0418551492644497, -345.0759160607198055 ) ) ;
#51264=CARTESIAN_POINT ( 'NONE',  ( 9.380405744046012018, -300.0735365612985106, -196.7602862293037731 ) ) ;
#51265=CARTESIAN_POINT ( 'NONE',  ( -92.27375911077636772, -282.8731231115476135, -323.9828403407423707 ) ) ;
#51266=CARTESIAN_POINT ( 'NONE',  ( 21.17220360774945220, -289.9420375074424783, -315.7037947314042299 ) ) ;
#51267=CARTESIAN_POINT ( 'NONE',  ( -33.39872607132846838, -299.6207851031292648, -194.0534482888731702 ) ) ;
#51268=CARTESIAN_POINT ( 'NONE',  ( -111.2431119366072352, -298.0133092692187802, -250.0008861325090379 ) ) ;
#51269=CARTESIAN_POINT ( 'NONE',  ( -5.973799624531089592, -296.6390399610475583, -338.3028816361386362 ) ) ;
#51270=CARTESIAN_POINT ( 'NONE',  ( -12.95540827744081191, -280.7345018623467467, -341.1644693185671713 ) ) ;
#51271=CARTESIAN_POINT ( 'NONE',  ( 10.55947360335228602, -272.7372355019858787, -213.0454916812439876 ) ) ;
#51272=CARTESIAN_POINT ( 'NONE',  ( -73.25418718593287792, -287.1845969734122832, -203.0960214877770795 ) ) ;
#51273=CARTESIAN_POINT ( 'NONE',  ( -13.19899063299152608, -287.6513335046544739, -339.5807369613722813 ) ) ;
#51274=CARTESIAN_POINT ( 'NONE',  ( -46.75580690834000563, -155.7037500639930556, -364.9887862212212326 ) ) ;
#51276=CARTESIAN_POINT ( 'NONE',  ( -72.91576878434101161, -288.0887723416465178, -338.0004029801337992 ) ) ;
#51277=CARTESIAN_POINT ( 'NONE',  ( -18.47213173214542792, -288.4691351571925679, -340.9546770565488032 ) ) ;
#51279=CARTESIAN_POINT ( 'NONE',  ( -108.7457342867439252, -285.9895661006634668, -242.2352704080417141 ) ) ;
#51280=CARTESIAN_POINT ( 'NONE',  ( -8.726480681712610377, -277.0004240130094217, -337.5554410759777966 ) ) ;
#51281=CARTESIAN_POINT ( 'NONE',  ( 27.83593559519302474, -293.0043085922339401, -310.8758121720233021 ) ) ;
#51282=CARTESIAN_POINT ( 'NONE',  ( 38.15303266288361073, -282.0204279340560447, -255.7372297268021271 ) ) ;
#51283=CARTESIAN_POINT ( 'NONE',  ( 38.18778090552909532, -283.2093621946389703, -281.2241400026125575 ) ) ;
#51284=CARTESIAN_POINT ( 'NONE',  ( 0.8615533933342958139, -282.8903013607180128, -337.2063973570359963 ) ) ;
#51286=CARTESIAN_POINT ( 'NONE',  ( -34.31670010331186660, -280.4244747725265370, -197.3901109744372206 ) ) ;
#51287=CARTESIAN_POINT ( 'NONE',  ( -77.71228223721278994, -208.7304540725825746, -357.2837420577297962 ) ) ;
#51288=CARTESIAN_POINT ( 'NONE',  ( -110.2672532426750394, -280.3355224829630288, -287.2074681069486246 ) ) ;
#51289=CARTESIAN_POINT ( 'NONE',  ( 152.7083132524945199, 207.2806415074720690, -216.8349236652551895 ) ) ;
#51290=CARTESIAN_POINT ( 'NONE',  ( -23.05802698232256276, -108.1619730152996510, -359.3355512241282099 ) ) ;
#51291=CARTESIAN_POINT ( 'NONE',  ( -29.96343797951733734, -273.3450898377187173, -197.5726369257234296 ) ) ;
#51292=CARTESIAN_POINT ( 'NONE',  ( 38.29559869269915851, -293.2370527439210264, -284.5221967548640123 ) ) ;
#51293=CARTESIAN_POINT ( 'NONE',  ( -54.63958497508173906, -170.0083358554137760, -360.9089503003181107 ) ) ;
#51294=CARTESIAN_POINT ( 'NONE',  ( 4.606858296998139757, -273.2900389422306375, -206.3168755091394075 ) ) ;
#51295=CARTESIAN_POINT ( 'NONE',  ( -56.29044453690115546, -287.7001020515376126, -341.7401652616800334 ) ) ;
#51296=CARTESIAN_POINT ( 'NONE',  ( -85.25760938254116184, -297.5822589470674870, -327.1289543838508393 ) ) ;
#51297=CARTESIAN_POINT ( 'NONE',  ( -31.81768368539835024, -290.2963063946691022, -343.6973392395946689 ) ) ;
#51298=ORIENTED_EDGE ( 'NONE', *, *, #40194, .T. ) ;
#51299=CARTESIAN_POINT ( 'NONE',  ( -66.82295980787920087, -296.3703552800276384, -341.2531668934860249 ) ) ;
#51300=CARTESIAN_POINT ( 'NONE',  ( -19.80715333753590812, -286.7760857790582349, -199.4349020232345993 ) ) ;
#51301=CARTESIAN_POINT ( 'NONE',  ( -64.77660902420062428, -272.6224856830560270, -198.7312219740244643 ) ) ;
#51302=CARTESIAN_POINT ( 'NONE',  ( 34.30854149943613862, -294.0009565589429030, -242.4580193273854434 ) ) ;
#51303=CARTESIAN_POINT ( 'NONE',  ( 37.40172060872340865, -294.2735517855292073, -288.6631250977949321 ) ) ;
#51304=CARTESIAN_POINT ( 'NONE',  ( -81.73072800137975946, -291.5953493553906810, -212.3435988334819911 ) ) ;
#51307=CARTESIAN_POINT ( 'NONE',  ( -106.7643302014827924, -274.8610345231431324, -240.3989706573248384 ) ) ;
#51308=CARTESIAN_POINT ( 'NONE',  ( 39.30990417282686877, -274.3574070850378348, -271.1827802559762972 ) ) ;
#51310=CARTESIAN_POINT ( 'NONE',  ( -97.64475288401712305, -278.6997196782659785, -222.5796494837631201 ) ) ;
#51311=CARTESIAN_POINT ( 'NONE',  ( -19.05388863936206434, -272.6911939619357099, -198.8098863554541254 ) ) ;
#51312=CARTESIAN_POINT ( 'NONE',  ( -72.06623429421867399, -274.6615927930545240, -205.7411494700859578 ) ) ;
#51313=CARTESIAN_POINT ( 'NONE',  ( -19.22497150002561028, -275.2321654090210927, -199.3494330304375239 ) ) ;
#51314=CARTESIAN_POINT ( 'NONE',  ( 18.63627104344689300, -300.3420462640792721, -194.1461562402953689 ) ) ;
#51315=CARTESIAN_POINT ( 'NONE',  ( 21.34383611093550925, -274.2198598528069056, -317.6511144384777481 ) ) ;
#51316=CARTESIAN_POINT ( 'NONE',  ( -82.41615070157540401, -296.3374367231871815, -327.9772502772240159 ) ) ;
#51317=CARTESIAN_POINT ( 'NONE',  ( -9.020755267232376085, -293.2490940668136545, -338.2961025804175961 ) ) ;
#51319=CARTESIAN_POINT ( 'NONE',  ( -11.88062928749293157, -277.2218893912382782, -343.0204507072509728 ) ) ;
#51320=CARTESIAN_POINT ( 'NONE',  ( -27.29227955308186537, -274.3499687997675665, -198.0052463807687957 ) ) ;
#51321=CARTESIAN_POINT ( 'NONE',  ( -113.8621955474651060, -283.2060724927833348, -272.8165877493603375 ) ) ;
#51322=CARTESIAN_POINT ( 'NONE',  ( -67.46745545333388350, -297.4465505707994453, -339.2266920765391092 ) ) ;
#51324=CARTESIAN_POINT ( 'NONE',  ( -2.099643807327661538, -285.7282144306698228, -206.1903179535610207 ) ) ;
#51326=CARTESIAN_POINT ( 'NONE',  ( -111.3638953955564546, -276.8246514181016096, -267.8518529840685005 ) ) ;
#51327=CARTESIAN_POINT ( 'NONE',  ( -109.6254634277432700, -276.9454204025141735, -284.2275108900748251 ) ) ;
#51328=CARTESIAN_POINT ( 'NONE',  ( -109.5792553573367343, -286.2923252711419764, -290.5759471552039486 ) ) ;
#51329=CARTESIAN_POINT ( 'NONE',  ( -8.830680336366494743, -275.6385956928988890, -202.6737006584762071 ) ) ;
#51331=CARTESIAN_POINT ( 'NONE',  ( 34.97723848205466624, -273.6447393864390847, -246.1860825442317662 ) ) ;
#51332=CARTESIAN_POINT ( 'NONE',  ( -61.48350515421354601, -281.7395822199710551, -199.1219377857263737 ) ) ;
#51335=CARTESIAN_POINT ( 'NONE',  ( 22.70197244248242896, -288.8488033283720142, -224.4697524299036502 ) ) ;
#51336=CARTESIAN_POINT ( 'NONE',  ( 27.32275329823826837, -292.0609984471067264, -308.4552361473316182 ) ) ;
#51338=CARTESIAN_POINT ( 'NONE',  ( -58.00193527136787708, -296.5741332006574567, -199.9318258683461806 ) ) ;
#51339=CARTESIAN_POINT ( 'NONE',  ( -63.20931109326946284, -289.8511557346079712, -200.7785613824553650 ) ) ;
#51340=CARTESIAN_POINT ( 'NONE',  ( 168.1488725781630649, 234.1813984995739588, -193.4213935641190858 ) ) ;
#51342=CARTESIAN_POINT ( 'NONE',  ( -74.11037536823270955, -288.0114460422887532, -337.2398715936250824 ) ) ;
#51343=CARTESIAN_POINT ( 'NONE',  ( 12.47151682149915786, -283.9442536367162120, -324.8137013068803185 ) ) ;
#51344=CARTESIAN_POINT ( 'NONE',  ( -32.35029913124321865, -284.3541113851138107, -194.5255695087189167 ) ) ;
#51345=EDGE_CURVE ( 'NONE', #30942, #56563, #16200, .T. ) ;
#51346=CARTESIAN_POINT ( 'NONE',  ( 1.427036243123854575, -283.9487498538712771, -332.9694892035441853 ) ) ;
#51347=CARTESIAN_POINT ( 'NONE',  ( -110.4710336452073989, -285.3835324466729730, -268.1926379186728582 ) ) ;
#51348=CARTESIAN_POINT ( 'NONE',  ( -99.31326752228548571, -291.9534794869913412, -313.2322229163359566 ) ) ;
#51349=AXIS2_PLACEMENT_3D ( 'NONE', #70832, #4547, #11651 ) ;
#51350=CARTESIAN_POINT ( 'NONE',  ( -76.42564679772937097, -273.8780621880021613, -203.9806774624228183 ) ) ;
#51351=CARTESIAN_POINT ( 'NONE',  ( -64.94420504085373125, -287.4896187115740531, -340.7542856627702577 ) ) ;
#51352=CARTESIAN_POINT ( 'NONE',  ( 39.62341770031462573, -275.5982112438683771, -274.0439643318902654 ) ) ;
#51354=CARTESIAN_POINT ( 'NONE',  ( -8.574200426926870122, -296.6537085379361542, -339.2537505169716496 ) ) ;
#51356=CARTESIAN_POINT ( 'NONE',  ( 21.31550574532285580, -296.6948066931273615, -317.0979686699210447 ) ) ;
#51357=CARTESIAN_POINT ( 'NONE',  ( -38.91229977634652215, -281.7570514290203505, -343.8500613152575056 ) ) ;
#51358=CARTESIAN_POINT ( 'NONE',  ( -97.35543649558452728, -275.9343644715334563, -315.6412824194929385 ) ) ;
#51359=CARTESIAN_POINT ( 'NONE',  ( -78.45158725841787373, -271.9893862814429895, -206.0751558145414322 ) ) ;
#51360=CARTESIAN_POINT ( 'NONE',  ( 22.36887989861714843, -274.3126577192658146, -228.1667141005777353 ) ) ;
#51361=CARTESIAN_POINT ( 'NONE',  ( -7.002322054124368478, -293.9778007656896079, -203.2028728277592506 ) ) ;
#51362=CARTESIAN_POINT ( 'NONE',  ( 33.34695230240954800, -294.7460569882038612, -289.5536156726855666 ) ) ;
#51363=CARTESIAN_POINT ( 'NONE',  ( -75.25822012815351059, -287.2993804090584149, -206.7976731066611933 ) ) ;
#51364=CARTESIAN_POINT ( 'NONE',  ( 36.84547423152254453, -294.7467286616699766, -252.0616793162862450 ) ) ;
#51365=CARTESIAN_POINT ( 'NONE',  ( 32.97001352374171290, -295.2554385341416037, -300.6539121235078937 ) ) ;
#51366=CARTESIAN_POINT ( 'NONE',  ( -90.40869541044028779, -295.6627419143641191, -320.5626925475636426 ) ) ;
#51367=CARTESIAN_POINT ( 'NONE',  ( -64.52259417479709214, -291.4069716192421993, -340.3181356888530900 ) ) ;
#51368=CARTESIAN_POINT ( 'NONE',  ( -63.91002463949956081, -283.5559343855917973, -342.6323026771391937 ) ) ;
#51369=CARTESIAN_POINT ( 'NONE',  ( -98.55485888375768866, -271.2949951125382313, -225.6282772434913682 ) ) ;
#51370=CARTESIAN_POINT ( 'NONE',  ( 7.545653922764927302, -286.4788797298362510, -207.7324745035944318 ) ) ;
#51371=CARTESIAN_POINT ( 'NONE',  ( -108.6812842002432404, -280.2454704615338414, -292.5001271597886330 ) ) ;
#51372=CARTESIAN_POINT ( 'NONE',  ( -72.55108138684782659, -284.3699796257046728, -205.9462821791904048 ) ) ;
#51373=CARTESIAN_POINT ( 'NONE',  ( 19.05180765752198369, -286.2390077329460496, -319.8251025343561764 ) ) ;
#51374=CARTESIAN_POINT ( 'NONE',  ( -14.57596635432840237, -278.4835867449974671, -198.0425159834175588 ) ) ;
#51375=CARTESIAN_POINT ( 'NONE',  ( -114.4693872376281121, -273.8646567567205921, -270.3778293100139649 ) ) ;
#51376=CARTESIAN_POINT ( 'NONE',  ( -71.20117712068562810, -285.1000708925562890, -205.6191357793204304 ) ) ;
#51377=CARTESIAN_POINT ( 'NONE',  ( 36.10240885156724744, -283.0338500426178143, -292.3146140444306411 ) ) ;
#51378=CARTESIAN_POINT ( 'NONE',  ( -93.42910324097664443, -288.8933169988201257, -322.8497945501792401 ) ) ;
#51379=CARTESIAN_POINT ( 'NONE',  ( 0.6658735846956594928, -278.1547510787144688, -336.4653906778946180 ) ) ;
#51380=CARTESIAN_POINT ( 'NONE',  ( -38.52045723407346145, -278.3818106649574702, -346.8588879259321516 ) ) ;
#51381=CARTESIAN_POINT ( 'NONE',  ( -32.96089309463820882, -279.9421988014126441, -197.4926849388189680 ) ) ;
#51382=CARTESIAN_POINT ( 'NONE',  ( -62.60966605852549804, -275.7015885356250351, -200.1231175860255860 ) ) ;
#51383=CARTESIAN_POINT ( 'NONE',  ( 39.22612934283546338, -293.4441570845385741, -261.7259186998205678 ) ) ;
#51384=CARTESIAN_POINT ( 'NONE',  ( -59.19420209856912152, -287.3563384424054448, -341.7895882359574102 ) ) ;
#51385=CARTESIAN_POINT ( 'NONE',  ( -4.962778673954555408, -294.0715167717559666, -201.3825280875441308 ) ) ;
#51386=CARTESIAN_POINT ( 'NONE',  ( 33.74243774670213725, -292.7080384216546918, -288.2851637620581187 ) ) ;
#51387=CARTESIAN_POINT ( 'NONE',  ( -34.30456222466462890, -294.6796352118220170, -343.3190735473191921 ) ) ;
#51388=CARTESIAN_POINT ( 'NONE',  ( -114.0806652775742265, -291.6207988044860144, -271.2389971882222994 ) ) ;
#51389=CARTESIAN_POINT ( 'NONE',  ( 30.11236519062958905, -281.8261398450110846, -242.1859207362689119 ) ) ;
#51390=CARTESIAN_POINT ( 'NONE',  ( -83.42922628208066271, -272.4967088667843882, -208.9043682662539254 ) ) ;
#51391=CARTESIAN_POINT ( 'NONE',  ( -9.592366059720150773, -289.3503335277848123, -342.0778332262464119 ) ) ;
#51392=CARTESIAN_POINT ( 'NONE',  ( -16.50465898389557751, -280.9254217157837843, -343.2586523003407137 ) ) ;
#51394=CARTESIAN_POINT ( 'NONE',  ( -23.31162333636806494, -289.2108809321733247, -346.1047236308979791 ) ) ;
#51395=CARTESIAN_POINT ( 'NONE',  ( -54.76549701512190182, -286.1553782475880325, -199.3968956021237204 ) ) ;
#51396=DIRECTION ( 'NONE',  ( 0.000000000000000000, 0.000000000000000000, 1.000000000000000000 ) ) ;
#51397=CARTESIAN_POINT ( 'NONE',  ( -23.56101253494735204, -107.7048510163219390, -360.7984423213250693 ) ) ;
#51398=CARTESIAN_POINT ( 'NONE',  ( 84.33524000671648935, 81.64880898236285134, -298.7293534775860735 ) ) ;
#51399=CARTESIAN_POINT ( 'NONE',  ( -67.36322160390778890, -278.8452327614540422, -203.6293444107159587 ) ) ;
#51400=CARTESIAN_POINT ( 'NONE',  ( -81.01450109818662781, -276.5816164338935437, -329.2416115957188367 ) ) ;
#51401=CARTESIAN_POINT ( 'NONE',  ( -52.53729328442921798, -273.5294786642951408, -194.8425405212830412 ) ) ;
#51402=CARTESIAN_POINT ( 'NONE',  ( 180.9896740030162334, 251.1209438834910941, -164.8178949726211044 ) ) ;
#51403=CARTESIAN_POINT ( 'NONE',  ( -101.3873539498802785, -277.6795321963437004, -228.5909497609535777 ) ) ;
#51404=CARTESIAN_POINT ( 'NONE',  ( -67.24105069211334751, -281.4662213769327082, -338.7699945286641992 ) ) ;
#51405=CARTESIAN_POINT ( 'NONE',  ( -22.27624258869237295, -296.6218995080958507, -344.8393429914403896 ) ) ;
#51406=CARTESIAN_POINT ( 'NONE',  ( -66.59446684659742743, -292.1506748908980740, -203.4114049053566191 ) ) ;
#51407=CARTESIAN_POINT ( 'NONE',  ( -71.41618139399894005, -288.1968084978206548, -335.4919496959481080 ) ) ;
#51408=CARTESIAN_POINT ( 'NONE',  ( -64.87134762020566825, -274.3532910164384475, -198.5456182762580397 ) ) ;
#51409=CARTESIAN_POINT ( 'NONE',  ( -77.51374711841455678, -297.6634811330434331, -209.3478787528440535 ) ) ;
#51412=CARTESIAN_POINT ( 'NONE',  ( -45.14935909155659743, -281.8742948270440820, -195.1535817487443580 ) ) ;
#51414=CARTESIAN_POINT ( 'NONE',  ( -22.14369121652733696, -281.3309695277396827, -198.5926110428148093 ) ) ;
#51415=CARTESIAN_POINT ( 'NONE',  ( -92.58171691235297374, -279.5895982078021689, -322.6143171171322592 ) ) ;
#51417=CARTESIAN_POINT ( 'NONE',  ( 35.75544495413252832, -280.5517729176612534, -265.8649164330307713 ) ) ;
#51418=CARTESIAN_POINT ( 'NONE',  ( -59.66743547012691806, -272.2376801242465376, -200.0775824269973384 ) ) ;
#51421=CARTESIAN_POINT ( 'NONE',  ( 37.75005991015741813, -276.5599169703956477, -286.7133135149941268 ) ) ;
#51422=CARTESIAN_POINT ( 'NONE',  ( 36.93973550371305237, -277.4193302799413345, -260.0040445923528978 ) ) ;
#51423=CARTESIAN_POINT ( 'NONE',  ( -112.2198929560257739, -276.9341662533229282, -285.6528870379738123 ) ) ;
#51426=CARTESIAN_POINT ( 'NONE',  ( 29.62718709690886598, -283.9870730079629197, -304.9092719664535025 ) ) ;
#51427=CARTESIAN_POINT ( 'NONE',  ( -67.85924666746414857, -290.8382078271920932, -203.8546398804367641 ) ) ;
#51428=CARTESIAN_POINT ( 'NONE',  ( 39.25393064353939820, -286.8082484606679827, -262.9753143014479519 ) ) ;
#51430=CARTESIAN_POINT ( 'NONE',  ( -18.49899670153819287, -281.0460798014408965, -341.9888668150459239 ) ) ;
#51431=CARTESIAN_POINT ( 'NONE',  ( -95.59390966811150747, -282.4986398064423270, -315.3489596925234082 ) ) ;
#51432=CARTESIAN_POINT ( 'NONE',  ( 30.38200422305712323, -282.3797132356800148, -242.0657054077556154 ) ) ;
#51433=CARTESIAN_POINT ( 'NONE',  ( -84.52961589271976095, -271.4021107443734877, -212.0661675029861613 ) ) ;
#51434=CARTESIAN_POINT ( 'NONE',  ( -93.82004815023677224, -282.2497098719531436, -321.5335470610789343 ) ) ;
#51435=CARTESIAN_POINT ( 'NONE',  ( -93.14597332543328889, -297.8540675974251144, -320.4889635898066444 ) ) ;
#51436=CARTESIAN_POINT ( 'NONE',  ( -106.4823877096816886, -279.1714356761793283, -294.6596929520679282 ) ) ;
#51437=CARTESIAN_POINT ( 'NONE',  ( -100.9801976548508833, -287.0888725472586316, -230.3589923139726068 ) ) ;
#51440=CARTESIAN_POINT ( 'NONE',  ( 35.71074242522526276, -295.7185769415397658, -289.6653879129536904 ) ) ;
#51441=CARTESIAN_POINT ( 'NONE',  ( 33.13256286020257591, -273.8865216935262197, -296.1707854824464334 ) ) ;
#51442=CARTESIAN_POINT ( 'NONE',  ( 0.6305773313442843975, -287.7568422106557477, -337.2214274436521464 ) ) ;
#51443=CARTESIAN_POINT ( 'NONE',  ( 2.691392010305296623, -290.9983933267406542, -208.3022497218942419 ) ) ;
#51444=CARTESIAN_POINT ( 'NONE',  ( -67.01704250314124067, -276.1343115458083162, -337.5966557142100442 ) ) ;
#51445=CARTESIAN_POINT ( 'NONE',  ( -110.1000124254166366, -294.4997796230364315, -285.1586130065427369 ) ) ;
#51446=CARTESIAN_POINT ( 'NONE',  ( -77.53879578183138221, -292.8153249138662204, -208.8352130454967437 ) ) ;
#51447=CARTESIAN_POINT ( 'NONE',  ( -37.30987171927208124, -279.5519495502701943, -345.3611179825600175 ) ) ;
#51448=CARTESIAN_POINT ( 'NONE',  ( -16.71309073743227458, -293.2703998742069871, -343.8812709142250696 ) ) ;
#51449=CARTESIAN_POINT ( 'NONE',  ( 34.48425296021367359, -288.9303289733669544, -253.3515399664831307 ) ) ;
#51450=CARTESIAN_POINT ( 'NONE',  ( -102.9351757981450532, -288.2849323774306640, -308.8249880105770444 ) ) ;
#51452=CARTESIAN_POINT ( 'NONE',  ( -20.98082687442135708, -290.2633378636901398, -342.1085690995844288 ) ) ;
#51454=CARTESIAN_POINT ( 'NONE',  ( -68.81820771131771153, -290.2797560707646198, -336.4052789502438827 ) ) ;
#51456=CARTESIAN_POINT ( 'NONE',  ( 20.28437933050187425, -289.4437260866753263, -320.8511097140428774 ) ) ;
#51457=CARTESIAN_POINT ( 'NONE',  ( -109.7496430750738483, -276.8396252520901726, -249.4925626328013948 ) ) ;
#51458=CARTESIAN_POINT ( 'NONE',  ( -38.17393650028858332, -280.3752688410053793, -193.3867607311133554 ) ) ;
#51460=CARTESIAN_POINT ( 'NONE',  ( -71.22146339282159033, -279.2837893561733722, -201.2387197835106463 ) ) ;
#51461=CARTESIAN_POINT ( 'NONE',  ( 32.33400821136631720, -285.9150837605819220, -298.2552784806180739 ) ) ;
#51463=CARTESIAN_POINT ( 'NONE',  ( -95.74823965925392599, -277.3272824979381994, -224.5199116817613572 ) ) ;
#51464=CARTESIAN_POINT ( 'NONE',  ( -82.69459577496682812, -281.6714023057865575, -330.1600784574403065 ) ) ;
#51465=DIRECTION ( 'NONE',  ( 0.9951408606192332362, 1.205805641958552022E-17, 0.09846150276129254919 ) ) ;
#51466=CARTESIAN_POINT ( 'NONE',  ( -88.45257126145590121, -277.8307061036803702, -213.7008443938491666 ) ) ;
#51467=CARTESIAN_POINT ( 'NONE',  ( -107.6372678634031956, -283.8664351519456091, -239.5685517524192676 ) ) ;
#51468=CARTESIAN_POINT ( 'NONE',  ( -89.36415982661537782, -274.0989427967181769, -218.9192535745787325 ) ) ;
#51469=CARTESIAN_POINT ( 'NONE',  ( -9.351672897702075105, -299.7108510549784341, -193.8481552504320859 ) ) ;
#51470=CARTESIAN_POINT ( 'NONE',  ( 28.04754862254848291, -275.6608127046996515, -302.9763796356857029 ) ) ;
#51471=CARTESIAN_POINT ( 'NONE',  ( 15.74957097491475722, -296.3011702534035408, -323.4088545178870504 ) ) ;
#51472=CARTESIAN_POINT ( 'NONE',  ( 0.7211415310280909763, -288.7261983510460936, -337.3558177322461802 ) ) ;
#51473=CARTESIAN_POINT ( 'NONE',  ( 34.80811009731442596, -279.3446851516665106, -247.9174310598610305 ) ) ;
#51474=CARTESIAN_POINT ( 'NONE',  ( -2.053946846237938217, -292.3396013615513880, -201.9082332835468776 ) ) ;
#51476=CARTESIAN_POINT ( 'NONE',  ( -29.15869370762009183, -288.0046506885831263, -343.1378096759977439 ) ) ;
#51477=CARTESIAN_POINT ( 'NONE',  ( 37.50432874118308035, -291.6233253216327626, -275.9170354931635529 ) ) ;
#51480=CARTESIAN_POINT ( 'NONE',  ( -109.4808660694708919, -289.9062295050376861, -282.0126272586754794 ) ) ;
#51482=CARTESIAN_POINT ( 'NONE',  ( 22.80004149195270458, -287.8528267523544741, -222.6349184610621990 ) ) ;
#51483=CARTESIAN_POINT ( 'NONE',  ( -82.13390479932378696, -287.9090924074130839, -214.2458315076590907 ) ) ;
#51484=CARTESIAN_POINT ( 'NONE',  ( -22.15585142638321869, -293.9209410872509807, -345.6087771587921225 ) ) ;
#51485=CARTESIAN_POINT ( 'NONE',  ( -8.211044061489817025, -283.9938639573693422, -341.1612280169849782 ) ) ;
#51486=CARTESIAN_POINT ( 'NONE',  ( -57.39234806562222246, -285.6195142118892250, -200.1161158421914763 ) ) ;
#51487=CARTESIAN_POINT ( 'NONE',  ( 33.32962563312794657, -276.6002865124329446, -250.0099622126104464 ) ) ;
#51488=CARTESIAN_POINT ( 'NONE',  ( 4.722953411414295033, -292.5011172347317370, -332.0248165667503599 ) ) ;
#51489=CARTESIAN_POINT ( 'NONE',  ( 7.586010280570228304, -273.4760008703399308, -212.3212063608265794 ) ) ;
#51491=CARTESIAN_POINT ( 'NONE',  ( -96.12512592106646991, -239.9971452530988358, -342.0757611934672582 ) ) ;
#51492=CARTESIAN_POINT ( 'NONE',  ( -32.01821008745215380, -294.6534699819620755, -347.1689308397690183 ) ) ;
#51493=CARTESIAN_POINT ( 'NONE',  ( -11.54545232377714470, -288.3109337429892776, -200.5337036185871682 ) ) ;
#51494=CARTESIAN_POINT ( 'NONE',  ( -110.9149370818568059, -297.3586985871093589, -292.0516070652091685 ) ) ;
#51495=CARTESIAN_POINT ( 'NONE',  ( 35.09599560119829675, -288.0691792901280905, -260.1594505518147571 ) ) ;
#51496=CARTESIAN_POINT ( 'NONE',  ( -98.62285123107045592, -276.9931017054823315, -316.6151600833169937 ) ) ;
#51497=CARTESIAN_POINT ( 'NONE',  ( 33.32617774255534471, -294.5917845606924743, -300.8166419520252930 ) ) ;
#51498=CARTESIAN_POINT ( 'NONE',  ( 13.75294810023830472, -286.4850339426432129, -326.3753983022115790 ) ) ;
#51499=CARTESIAN_POINT ( 'NONE',  ( 0.5337987675556906675, -294.8949596031568490, -337.3926416029415805 ) ) ;
#51500=CARTESIAN_POINT ( 'NONE',  ( -17.43090634539850825, -292.6493979765727431, -200.0543458388402485 ) ) ;
#51503=CARTESIAN_POINT ( 'NONE',  ( -93.16763214118681447, -239.2410508537433884, -338.7284373407006797 ) ) ;
#51504=CARTESIAN_POINT ( 'NONE',  ( 21.54268577276647179, -288.4142508919589432, -221.8293051974474110 ) ) ;
#51505=CARTESIAN_POINT ( 'NONE',  ( -99.90806341382575795, -281.4094976428775112, -320.2154176792147382 ) ) ;
#51507=CARTESIAN_POINT ( 'NONE',  ( -22.57761245057275801, -279.5848302304230515, -194.8394933818699428 ) ) ;
#51508=CARTESIAN_POINT ( 'NONE',  ( 28.04878311192764428, -283.0669582122817474, -233.9727527325047447 ) ) ;
#51509=CARTESIAN_POINT ( 'NONE',  ( 181.7656723149513880, 252.4586733329624053, -166.1422410563588130 ) ) ;
#51510=CARTESIAN_POINT ( 'NONE',  ( -68.24568264764472758, -284.2289048048329505, -200.4644511332673744 ) ) ;
#51511=CARTESIAN_POINT ( 'NONE',  ( 17.04668346832513848, -286.3495989613521147, -321.2618796214046597 ) ) ;
#51512=CARTESIAN_POINT ( 'NONE',  ( -46.75145511815055244, -275.7943065919627088, -195.1829164207212557 ) ) ;
#51513=CARTESIAN_POINT ( 'NONE',  ( -84.11903992990953327, -297.8813703588620569, -214.1713655441783999 ) ) ;
#51514=CARTESIAN_POINT ( 'NONE',  ( 8.522949523767147539, -293.0939367030430276, -327.8519173053024929 ) ) ;
#51515=CARTESIAN_POINT ( 'NONE',  ( -67.66077212544553277, -278.0910863022785975, -341.0298285978793729 ) ) ;
#51516=CARTESIAN_POINT ( 'NONE',  ( 29.15426609100027378, -275.9581228753388018, -300.4823144493466884 ) ) ;
#51517=CARTESIAN_POINT ( 'NONE',  ( -102.2425666139509559, -278.3589462117289486, -236.6091812185341325 ) ) ;
#51518=CARTESIAN_POINT ( 'NONE',  ( 21.60441516583463084, -275.9692775008721242, -221.3014807778387478 ) ) ;
#51519=CARTESIAN_POINT ( 'NONE',  ( -5.426000899097470409, -275.5623375294906054, -340.0954757530493566 ) ) ;
#51520=CARTESIAN_POINT ( 'NONE',  ( -108.1563228279122768, -262.1275830946152041, -317.5270657317772702 ) ) ;
#51521=CARTESIAN_POINT ( 'NONE',  ( -46.06852554266539101, -275.1625392261226466, -344.9032639548833004 ) ) ;
#51523=CARTESIAN_POINT ( 'NONE',  ( -105.9919509934429698, -298.4115808985222316, -236.8089295680381952 ) ) ;
#51524=CARTESIAN_POINT ( 'NONE',  ( 31.95455697924148097, -277.6233781216988064, -236.9535640164627637 ) ) ;
#51525=CARTESIAN_POINT ( 'NONE',  ( -87.71122462277782006, -229.8683413793775117, -344.1918058839762011 ) ) ;
#51526=CARTESIAN_POINT ( 'NONE',  ( -6.900640255930542644, -287.5409829054607940, -203.6572456730689282 ) ) ;
#51527=CARTESIAN_POINT ( 'NONE',  ( -103.5232766187397999, -285.8201101801178652, -307.8035823936453994 ) ) ;
#51528=CARTESIAN_POINT ( 'NONE',  ( 6.995324597041635784, -286.0223298788998250, -212.1755509813080778 ) ) ;
#51529=CARTESIAN_POINT ( 'NONE',  ( -98.32121526661819644, -276.3799919904208764, -311.9296054340202886 ) ) ;
#51530=CARTESIAN_POINT ( 'NONE',  ( -76.76332396977754513, -285.4459938954857421, -333.3250083207291254 ) ) ;
#51531=CARTESIAN_POINT ( 'NONE',  ( -14.07176115676825034, -278.8392872868009817, -200.3842248877257646 ) ) ;
#51532=CARTESIAN_POINT ( 'NONE',  ( -39.15167158012825865, -278.1550714810845193, -343.6478840308668055 ) ) ;
#51534=CARTESIAN_POINT ( 'NONE',  ( -99.33600732362529584, -273.5776517489460957, -231.6998412713061555 ) ) ;
#51535=CARTESIAN_POINT ( 'NONE',  ( -17.04450508939578768, -281.1105946589420910, -196.2518561215067905 ) ) ;
#51536=CARTESIAN_POINT ( 'NONE',  ( 13.64470276825844230, -282.8529038051732982, -328.0507303541347710 ) ) ;
#51540=CARTESIAN_POINT ( 'NONE',  ( 38.12206254256724236, -289.3196729603439508, -263.0524668228799783 ) ) ;
#51541=CARTESIAN_POINT ( 'NONE',  ( -70.44097758174139301, -288.1641391424131484, -339.3518567632083887 ) ) ;
#51542=CARTESIAN_POINT ( 'NONE',  ( -106.1425256547889262, -295.4168378874039718, -295.3908183492602575 ) ) ;
#51543=CARTESIAN_POINT ( 'NONE',  ( -47.72141014014221838, -291.2722034441277970, -194.1130751415974203 ) ) ;
#51545=CARTESIAN_POINT ( 'NONE',  ( 28.84203366586359607, -286.4669256282139145, -302.7713190245626151 ) ) ;
#51546=CARTESIAN_POINT ( 'NONE',  ( 28.00470673309790826, -288.3042642937858204, -236.8278898279071427 ) ) ;
#51547=CARTESIAN_POINT ( 'NONE',  ( -114.2704648735229114, -299.0519495502701943, -270.3937649182068981 ) ) ;
#51548=CARTESIAN_POINT ( 'NONE',  ( 34.86597864598481777, -289.8137000892604647, -290.6826865948855811 ) ) ;
#51549=CARTESIAN_POINT ( 'NONE',  ( -95.87879206254001474, -287.9043026808990362, -317.5347622934455103 ) ) ;
#51551=CARTESIAN_POINT ( 'NONE',  ( -99.22345584756880044, -284.9527490412704651, -309.6230683398875385 ) ) ;
#51552=CARTESIAN_POINT ( 'NONE',  ( -97.74686961344146141, -293.1617239508714761, -225.6042820436836109 ) ) ;
#51555=CARTESIAN_POINT ( 'NONE',  ( -101.3358179605779981, -275.0639070193280986, -230.5721787613621530 ) ) ;
#51556=CARTESIAN_POINT ( 'NONE',  ( 34.64249328587163035, -280.9223010025953045, -283.5032802121699547 ) ) ;
#51557=CARTESIAN_POINT ( 'NONE',  ( -33.41634072821867818, -281.0025978053354834, -345.2712460209173173 ) ) ;
#51558=CARTESIAN_POINT ( 'NONE',  ( 39.44514265855386270, -292.7846346989077801, -273.1788466563999123 ) ) ;
#51559=CARTESIAN_POINT ( 'NONE',  ( -37.12704547263024324, -296.4547617808264590, -196.5582917753991694 ) ) ;
#51560=CARTESIAN_POINT ( 'NONE',  ( 36.26922387774162360, -273.4875589136615304, -259.1960850271480012 ) ) ;
#51561=CARTESIAN_POINT ( 'NONE',  ( -73.10138559252372659, -298.8826822098195066, -206.1545110475628917 ) ) ;
#51563=CARTESIAN_POINT ( 'NONE',  ( -57.94515094746591188, -272.3659471441075652, -196.7255249332656604 ) ) ;
#51564=CARTESIAN_POINT ( 'NONE',  ( -65.25243010132754762, -293.6518021448031277, -341.0502221943905283 ) ) ;
#51566=CARTESIAN_POINT ( 'NONE',  ( 34.35357825303041324, -295.1951546965901798, -287.0046998196123695 ) ) ;
#51568=CARTESIAN_POINT ( 'NONE',  ( -35.63662330301218617, -295.8330851369480570, -343.5152470036020986 ) ) ;
#51570=CARTESIAN_POINT ( 'NONE',  ( -111.5224520475220658, -282.3992386006758011, -283.9004205813481008 ) ) ;
#51571=CARTESIAN_POINT ( 'NONE',  ( -107.8356591662239055, -296.8031960251138912, -251.3497813343888936 ) ) ;
#51572=CARTESIAN_POINT ( 'NONE',  ( -87.74994165089476894, -285.3708314892757016, -212.0839224961861760 ) ) ;
#51573=CARTESIAN_POINT ( 'NONE',  ( 23.95374330326716716, -284.0695214465138179, -314.5666032461355144 ) ) ;
#51574=CARTESIAN_POINT ( 'NONE',  ( 9.801154225267605824, -286.3481616322209220, -209.5064092505764961 ) ) ;
#51575=CARTESIAN_POINT ( 'NONE',  ( -47.21167348868880964, -289.9262888767061099, -196.1815247602738452 ) ) ;
#51576=CARTESIAN_POINT ( 'NONE',  ( -111.3446827290143801, -277.6384391010379886, -291.2625857043049677 ) ) ;
#51577=CARTESIAN_POINT ( 'NONE',  ( -20.19161114001082069, -277.7666405000204009, -195.3683826091709363 ) ) ;
#51579=CARTESIAN_POINT ( 'NONE',  ( 35.39175343796056694, -286.2129898035755105, -260.1417195151675514 ) ) ;
#51580=CARTESIAN_POINT ( 'NONE',  ( -48.83629899556947862, -288.1154695846664708, -346.2394255820412923 ) ) ;
#51581=CARTESIAN_POINT ( 'NONE',  ( 133.0872704186301405, -299.5541904835127980, -195.3611179825600175 ) ) ;
#51582=CARTESIAN_POINT ( 'NONE',  ( -106.8904003388547466, -280.3864918002959712, -238.5858381513849622 ) ) ;
#51583=CARTESIAN_POINT ( 'NONE',  ( -37.70686698473414822, -293.0767806102421673, -345.7282360733721589 ) ) ;
#51584=CARTESIAN_POINT ( 'NONE',  ( 33.47712789946047707, -280.9834423564890926, -252.5119597210160407 ) ) ;
#51585=CARTESIAN_POINT ( 'NONE',  ( 37.09711093659996095, -293.9653863938079326, -290.0553661733474655 ) ) ;
#51586=CARTESIAN_POINT ( 'NONE',  ( -18.51669669479845126, -284.3725038957269931, -197.1296308933189607 ) ) ;
#51588=CARTESIAN_POINT ( 'NONE',  ( -108.7542917987817077, -280.2545261917697985, -293.4463161030702167 ) ) ;
#51589=CARTESIAN_POINT ( 'NONE',  ( -34.30339225811070492, -294.0717626604970292, -343.5333609022540600 ) ) ;
#51592=CARTESIAN_POINT ( 'NONE',  ( 20.94490568316089707, -282.8877125334589095, -223.7293864005971216 ) ) ;
#51593=CARTESIAN_POINT ( 'NONE',  ( -106.9298080458953564, -295.7629108594917966, -292.7844062299135430 ) ) ;
#51595=CARTESIAN_POINT ( 'NONE',  ( -95.99890600148557951, -281.4094976428775681, -317.0979686699210447 ) ) ;
#51596=CARTESIAN_POINT ( 'NONE',  ( 2.343374020077495068, -273.7668932137033835, -204.5640533806881365 ) ) ;
#51597=CARTESIAN_POINT ( 'NONE',  ( -110.3063956430286510, -290.3386970636212254, -273.9068405058119993 ) ) ;
#51598=CARTESIAN_POINT ( 'NONE',  ( -107.1073257192191335, -280.3866126434344892, -246.4668656059827470 ) ) ;
#51599=CARTESIAN_POINT ( 'NONE',  ( -57.09513368708623204, -275.3933308992231446, -199.2005607208959077 ) ) ;
#51600=CARTESIAN_POINT ( 'NONE',  ( -47.13317081521313412, -284.7746942242131354, -345.9294150123008080 ) ) ;
#51601=CARTESIAN_POINT ( 'NONE',  ( 34.72704160853412247, -280.1638233896074439, -256.3942250783815666 ) ) ;
#51602=CARTESIAN_POINT ( 'NONE',  ( -29.47910173162345515, -278.9528598568939515, -345.0001490536233177 ) ) ;
#51604=CARTESIAN_POINT ( 'NONE',  ( -64.89809936468039098, -273.5353297490814839, -198.4466900184550013 ) ) ;
#51605=CARTESIAN_POINT ( 'NONE',  ( -73.34443220093123728, -293.4913029372727351, -205.1486192212192066 ) ) ;
#51608=CARTESIAN_POINT ( 'NONE',  ( -11.50112392889963253, -292.8588402021799766, -341.6387504825224255 ) ) ;
#51609=CARTESIAN_POINT ( 'NONE',  ( 2.969114865619621568, -274.1168070937578705, -209.3660418895248370 ) ) ;
#51612=CARTESIAN_POINT ( 'NONE',  ( 27.45329504610856119, -294.5391058367924870, -229.9585084527130618 ) ) ;
#51613=CARTESIAN_POINT ( 'NONE',  ( -20.19161114001083490, -285.3376638359844719, -345.3538533559490702 ) ) ;
#51614=CARTESIAN_POINT ( 'NONE',  ( 22.78679633143006100, -294.1188887239611631, -222.8788878413000134 ) ) ;
#51615=CARTESIAN_POINT ( 'NONE',  ( 36.77972346564443029, -289.6860340952448496, -280.7523597154669233 ) ) ;
#51616=CARTESIAN_POINT ( 'NONE',  ( 14.99578389997540206, -274.3122857512170185, -323.9198584516471442 ) ) ;
#51618=CARTESIAN_POINT ( 'NONE',  ( 6.259644447126521349, -278.3756213712943577, -330.7591618347854592 ) ) ;
#51619=CARTESIAN_POINT ( 'NONE',  ( 37.08057606013549901, -291.6735687044987344, -273.5750589786385376 ) ) ;
#51620=CARTESIAN_POINT ( 'NONE',  ( -92.19609144501890796, -281.1393604072019912, -218.0242795429592775 ) ) ;
#51622=CARTESIAN_POINT ( 'NONE',  ( -8.489791802609559568, -282.3304788351815660, -337.4405848320453174 ) ) ;
#51623=CARTESIAN_POINT ( 'NONE',  ( -84.38819405829782738, -280.5017872345344472, -209.7288997785005051 ) ) ;
#51624=CARTESIAN_POINT ( 'NONE',  ( 32.02627016541798355, -280.7667768477475079, -302.9836265505269353 ) ) ;
#51625=CARTESIAN_POINT ( 'NONE',  ( -68.90763339293847878, -278.3983720020250416, -340.3498446071059220 ) ) ;
#51627=CARTESIAN_POINT ( 'NONE',  ( 25.56195184069837723, -276.4967306381847152, -227.1426158259065176 ) ) ;
#51628=CARTESIAN_POINT ( 'NONE',  ( -92.08974858914540107, -287.6948066931273047, -226.7417163044926838 ) ) ;
#51630=CARTESIAN_POINT ( 'NONE',  ( -99.37691940767398080, -275.1208352733501101, -228.4157905965967927 ) ) ;
#51631=CARTESIAN_POINT ( 'NONE',  ( -57.75414217784511806, -292.8620947905608887, -199.8980839639592091 ) ) ;
#51632=CARTESIAN_POINT ( 'NONE',  ( -43.36438112073825835, -275.1487065485370636, -344.7625569244016788 ) ) ;
#51633=CARTESIAN_POINT ( 'NONE',  ( -110.9349403241829464, -292.0717447851199609, -289.3342355719657917 ) ) ;
#51634=CARTESIAN_POINT ( 'NONE',  ( -38.89143457441620200, -291.3807856368616171, -197.2756133208389713 ) ) ;
#51635=CARTESIAN_POINT ( 'NONE',  ( 23.23512552972464107, -287.6945525438034679, -317.8162318287989478 ) ) ;
#51637=CARTESIAN_POINT ( 'NONE',  ( 38.27154246693870476, -291.9836314069960395, -258.9944522024007938 ) ) ;
#51638=CARTESIAN_POINT ( 'NONE',  ( -61.81907311342790479, -281.7753799530041761, -340.0374878636112612 ) ) ;
#51639=CARTESIAN_POINT ( 'NONE',  ( -111.0124639627065903, -292.2940468195929498, -279.4980778574630449 ) ) ;
#51640=CARTESIAN_POINT ( 'NONE',  ( -110.9191896322689104, -283.0968601607828532, -265.3994165696995537 ) ) ;
#51641=CARTESIAN_POINT ( 'NONE',  ( 33.92974531635276492, -282.6316308831800939, -252.3761424678914125 ) ) ;
#51642=CARTESIAN_POINT ( 'NONE',  ( -112.3329090950867197, -291.2875975136693683, -286.7665680445915086 ) ) ;
#51643=CARTESIAN_POINT ( 'NONE',  ( 35.09294997241880054, -281.9136679203530775, -260.4348292019039377 ) ) ;
#51644=CARTESIAN_POINT ( 'NONE',  ( -25.06985353031387120, -291.0002499313933413, -194.7475576992289064 ) ) ;
#51645=CARTESIAN_POINT ( 'NONE',  ( 1.431349676844140939, -287.3592656706775301, -204.0072160270258905 ) ) ;
#51646=CARTESIAN_POINT ( 'NONE',  ( 38.49513895880458136, -287.8811516476849874, -257.3105717182550052 ) ) ;
#51647=CARTESIAN_POINT ( 'NONE',  ( -33.24077978194360128, -286.2717666972439474, -197.4265775622738772 ) ) ;
#51650=CARTESIAN_POINT ( 'NONE',  ( -30.67564585599519589, -296.8291322073731635, -345.8321004901878268 ) ) ;
#51651=CARTESIAN_POINT ( 'NONE',  ( -32.06336046332013012, -293.6717356359525866, -346.6988407170836695 ) ) ;
#51652=CARTESIAN_POINT ( 'NONE',  ( -71.77538176415235682, -276.5777251577628135, -335.0106260483595406 ) ) ;
#51653=CARTESIAN_POINT ( 'NONE',  ( -75.72182459495267892, -296.9028726064447596, -203.6645925338374354 ) ) ;
#51654=CARTESIAN_POINT ( 'NONE',  ( 36.33429432913775514, -292.0735364145804738, -273.5379849549560163 ) ) ;
#51655=CARTESIAN_POINT ( 'NONE',  ( -105.6895157450809961, -295.1676507923224335, -241.9612920727463461 ) ) ;
#51656=CARTESIAN_POINT ( 'NONE',  ( 17.02200831704047701, -294.0537411095587572, -220.9741447264666476 ) ) ;
#51657=CARTESIAN_POINT ( 'NONE',  ( 29.01248043674391042, -294.2111676511165683, -239.0748898811623917 ) ) ;
#51659=CARTESIAN_POINT ( 'NONE',  ( -4.063910376749810816, -292.6142979405661890, -337.7743125028446229 ) ) ;
#51660=CARTESIAN_POINT ( 'NONE',  ( -99.18376716040198460, -297.9771256121612737, -312.8166145294829334 ) ) ;
#51661=CARTESIAN_POINT ( 'NONE',  ( -109.8542345570249950, -291.3572682127912117, -280.7145499118705629 ) ) ;
#51662=CARTESIAN_POINT ( 'NONE',  ( -9.218816181171575863, -295.0073634883732439, -337.7630868465290064 ) ) ;
#51663=CARTESIAN_POINT ( 'NONE',  ( -81.56029844326707234, -279.6305310699261213, -331.3785119213960684 ) ) ;
#51664=CARTESIAN_POINT ( 'NONE',  ( -33.92045886808352151, -278.7791807461813960, -193.9308008180744025 ) ) ;
#51665=VERTEX_POINT ( 'NONE', #64472 ) ;
#51666=CARTESIAN_POINT ( 'NONE',  ( -73.88909482989376443, -272.9287860919027366, -202.6439581546898125 ) ) ;
#51667=CARTESIAN_POINT ( 'NONE',  ( 18.67261079882158725, -280.3180480034368998, -319.3887751887700119 ) ) ;
#51668=CARTESIAN_POINT ( 'NONE',  ( -113.5847819481960101, -276.9366823302664216, -271.5751011180207115 ) ) ;
#51669=CARTESIAN_POINT ( 'NONE',  ( -83.42243452349075028, -277.4224509311123938, -210.9101312106916453 ) ) ;
#51670=CARTESIAN_POINT ( 'NONE',  ( -65.74796355123966407, -296.3574412365002786, -202.5796479696884944 ) ) ;
#51671=CARTESIAN_POINT ( 'NONE',  ( -112.3417001281054297, -274.5519904173220311, -270.3865538441530134 ) ) ;
#51674=CARTESIAN_POINT ( 'NONE',  ( -112.7228054487562758, -288.5976714566861574, -268.3724124827416517 ) ) ;
#51675=AXIS2_PLACEMENT_3D ( 'NONE', #25600, #69173, #38867 ) ;
#51676=CARTESIAN_POINT ( 'NONE',  ( -114.1124757261751483, -290.4697041760436491, -276.9535925488979160 ) ) ;
#51677=CARTESIAN_POINT ( 'NONE',  ( 3.836990852237445626, -276.6048393859001635, -207.4158012753741787 ) ) ;
#51678=CARTESIAN_POINT ( 'NONE',  ( -100.9639638295098507, -271.0855457997349163, -230.6470372420505441 ) ) ;
#51679=CARTESIAN_POINT ( 'NONE',  ( -37.97084460644526160, -285.2416296256656096, -193.5251693742420400 ) ) ;
#51682=CARTESIAN_POINT ( 'NONE',  ( -35.20354040728916800, -281.0251771647569967, -345.3432887154716013 ) ) ;
#51684=CARTESIAN_POINT ( 'NONE',  ( 13.18757191924456151, -291.5727708067083199, -217.1265129731111756 ) ) ;
#51685=CARTESIAN_POINT ( 'NONE',  ( -86.52711838184109183, -283.5003021195386737, -214.6897341499047513 ) ) ;
#51688=CARTESIAN_POINT ( 'NONE',  ( 35.25024326259225660, -291.3097428884024680, -251.5087863881390149 ) ) ;
#51689=CARTESIAN_POINT ( 'NONE',  ( -81.27951722050408989, -279.2609849072333645, -329.6562159443857354 ) ) ;
#51690=CARTESIAN_POINT ( 'NONE',  ( -3.056718355146273325, -283.8144285654549890, -338.8778774335357866 ) ) ;
#51691=CARTESIAN_POINT ( 'NONE',  ( -0.7215142817322897084, -272.6144445692577847, -204.2534669931673079 ) ) ;
#51692=CARTESIAN_POINT ( 'NONE',  ( -105.5649326430529271, -284.8989327378303642, -244.3882370255285252 ) ) ;
#51693=CARTESIAN_POINT ( 'NONE',  ( 27.14418845292203741, -276.4957481868808600, -234.8015397374245481 ) ) ;
#51694=CARTESIAN_POINT ( 'NONE',  ( 19.31311742701443279, -277.0091579537096891, -316.6716112503846716 ) ) ;
#51696=CARTESIAN_POINT ( 'NONE',  ( -110.2682972287494891, -286.3267434943717262, -287.9286054130099046 ) ) ;
#51699=CARTESIAN_POINT ( 'NONE',  ( -112.6056091699295791, -296.1821361037062843, -286.6197772223017068 ) ) ;
#51700=CARTESIAN_POINT ( 'NONE',  ( 12.20745792215177516, -288.7250639320607775, -214.4640308664372981 ) ) ;
#51702=CARTESIAN_POINT ( 'NONE',  ( -115.3430155898818299, -293.8380690714490129, -288.1317622949166548 ) ) ;
#51703=CARTESIAN_POINT ( 'NONE',  ( -56.46622564396024302, -278.7317438173255368, -196.0382793546128255 ) ) ;
#51704=CARTESIAN_POINT ( 'NONE',  ( -1.165508133930641899, -290.9238889895950138, -203.2960484647188082 ) ) ;
#51705=CARTESIAN_POINT ( 'NONE',  ( -65.37473102826832871, -287.1991883730297559, -202.1536045630575131 ) ) ;
#51706=CARTESIAN_POINT ( 'NONE',  ( -108.7927429910693320, -280.0607702022878129, -289.6671400754698311 ) ) ;
#51707=CARTESIAN_POINT ( 'NONE',  ( 28.40605071646576008, -289.4885580561158918, -309.2949021636125622 ) ) ;
#51708=CARTESIAN_POINT ( 'NONE',  ( 20.04056526586238718, -284.2201907275607482, -318.6747089409196292 ) ) ;
#51709=CARTESIAN_POINT ( 'NONE',  ( -111.3378347064482483, -278.9858507896692004, -249.0638864259610159 ) ) ;
#51710=CARTESIAN_POINT ( 'NONE',  ( -80.66259005203754384, -295.4813998916320656, -209.5733947463996856 ) ) ;
#51711=CARTESIAN_POINT ( 'NONE',  ( -114.3777617634478361, -278.4058452298719430, -268.7321277066191669 ) ) ;
#51712=CARTESIAN_POINT ( 'NONE',  ( -36.74962053950157781, -275.9200846893302810, -196.1156507256139037 ) ) ;
#51714=CARTESIAN_POINT ( 'NONE',  ( -54.49178911615187815, -288.3376638359845856, -195.3683826091709363 ) ) ;
#51715=CARTESIAN_POINT ( 'NONE',  ( -100.3555003455923895, -271.3600266310947973, -227.8029686674794618 ) ) ;
#51717=CARTESIAN_POINT ( 'NONE',  ( -64.83346329196058377, -279.1907823994736191, -202.6692322067896441 ) ) ;
#51718=CARTESIAN_POINT ( 'NONE',  ( 39.31022670569921473, -276.7671707211511034, -271.1521465307259859 ) ) ;
#51719=CARTESIAN_POINT ( 'NONE',  ( -24.58452265463143860, -281.9520499287045823, -346.1123236937039565 ) ) ;
#51720=CARTESIAN_POINT ( 'NONE',  ( -31.77304763926113651, -290.7412018032209176, -344.2159951128452349 ) ) ;
#51721=CARTESIAN_POINT ( 'NONE',  ( -30.58069267507421429, -299.6554609107259921, -194.0527348764640863 ) ) ;
#51722=CARTESIAN_POINT ( 'NONE',  ( -97.04656720098439848, -298.4037222275503041, -222.3680188080467701 ) ) ;
#51723=CARTESIAN_POINT ( 'NONE',  ( 15.63163035019207747, -296.3011702540286478, -323.2909306849135191 ) ) ;
#51724=CARTESIAN_POINT ( 'NONE',  ( 20.26327926962336434, -278.8910007609364357, -222.5741322981677399 ) ) ;
#51725=CARTESIAN_POINT ( 'NONE',  ( -27.03875510055579667, -272.2037422874089430, -196.3787248729832982 ) ) ;
#51726=CARTESIAN_POINT ( 'NONE',  ( -80.50203437437069454, -287.0782939394681534, -207.4991215171385477 ) ) ;
#51727=CARTESIAN_POINT ( 'NONE',  ( -86.94862462529601999, -288.6821678992318425, -324.4057227234073935 ) ) ;
#51728=CARTESIAN_POINT ( 'NONE',  ( 175.5833602167774075, 242.2213184666997847, -179.4617043395230382 ) ) ;
#51730=CARTESIAN_POINT ( 'NONE',  ( 0.4122403315564826531, -287.1345029591557818, -336.8531712378951397 ) ) ;
#51731=CARTESIAN_POINT ( 'NONE',  ( 31.41788371323971063, -287.5460617981311202, -294.9417428059152826 ) ) ;
#51733=CARTESIAN_POINT ( 'NONE',  ( -112.0616838708246803, -285.8487346899426598, -253.0863809110456373 ) ) ;
#51734=CARTESIAN_POINT ( 'NONE',  ( -76.36353307757454445, -277.9226512050869928, -332.1407914791986968 ) ) ;
#51735=CARTESIAN_POINT ( 'NONE',  ( 31.94483059854229268, -292.8969094194542890, -303.3614406634127363 ) ) ;
#51736=CARTESIAN_POINT ( 'NONE',  ( 24.17855000973035473, -282.8184109370029091, -316.4975635533658078 ) ) ;
#51737=CARTESIAN_POINT ( 'NONE',  ( 35.92850781740990840, -282.8020480421558887, -249.0027144860982276 ) ) ;
#51738=CARTESIAN_POINT ( 'NONE',  ( -88.30436075307106591, -284.0761832059829430, -328.1258884340070949 ) ) ;
#51739=CARTESIAN_POINT ( 'NONE',  ( -24.87695345809282799, -280.5488422214895650, -198.4117081368473805 ) ) ;
#51740=CARTESIAN_POINT ( 'NONE',  ( -95.95921662488163406, -270.6952119285918457, -223.5744983911110353 ) ) ;
#51741=CARTESIAN_POINT ( 'NONE',  ( -112.2661335305100607, -271.5905929391889231, -296.4060789002301703 ) ) ;
#51744=CARTESIAN_POINT ( 'NONE',  ( -71.26159565677255614, -279.5012423282600480, -337.0654590507153330 ) ) ;
#51745=CARTESIAN_POINT ( 'NONE',  ( 202.2090562182569329, 295.8239156117442690, -54.00000000003540634 ) ) ;
#51746=CARTESIAN_POINT ( 'NONE',  ( -48.83192253240383707, -154.4817910994489125, -361.7742097625079509 ) ) ;
#51748=CARTESIAN_POINT ( 'NONE',  ( -107.9319282003822025, -296.1518881054044527, -251.3152091021987928 ) ) ;
#51749=CARTESIAN_POINT ( 'NONE',  ( 17.51326807713136091, -293.8017528632220206, -324.3855614581157170 ) ) ;
#51750=CARTESIAN_POINT ( 'NONE',  ( -38.24214191940907881, -140.5200643640481530, -361.2081418523172260 ) ) ;
#51751=ADVANCED_FACE ( 'NONE', ( #13780 ), #72470, .F. ) ;
#51753=CARTESIAN_POINT ( 'NONE',  ( 18.86779562414340461, -297.3175958210166527, -193.9636422523521446 ) ) ;
#51754=CARTESIAN_POINT ( 'NONE',  ( -101.0042690261450389, -288.4438275629378268, -307.7916663922778753 ) ) ;
#51755=CARTESIAN_POINT ( 'NONE',  ( -67.78037544935655490, -297.3163264815419780, -338.0829004485497649 ) ) ;
#51757=CARTESIAN_POINT ( 'NONE',  ( -29.10131066803382538, -290.2607129870415861, -343.3908342571914432 ) ) ;
#51759=CARTESIAN_POINT ( 'NONE',  ( -24.93399507428794237, -295.8389866957581376, -346.1703434077252837 ) ) ;
#51760=CARTESIAN_POINT ( 'NONE',  ( -9.475717188045660322, -286.9187402820135162, -202.8089034423035457 ) ) ;
#51761=CARTESIAN_POINT ( 'NONE',  ( -40.40891024762056105, -296.8094625049994875, -193.7677614475972803 ) ) ;
#51762=CARTESIAN_POINT ( 'NONE',  ( -81.84519527958066476, -292.2655190776030167, -207.7224898098984340 ) ) ;
#51763=CARTESIAN_POINT ( 'NONE',  ( 1.663490251089023708, -293.0510353660948226, -203.9818970056705041 ) ) ;
#51764=CARTESIAN_POINT ( 'NONE',  ( -98.30070881451759135, -291.2769263791527123, -230.1071322280571394 ) ) ;
#51767=CARTESIAN_POINT ( 'NONE',  ( -63.08981177487974179, -275.6395554477534802, -199.3234593506664964 ) ) ;
#51768=CARTESIAN_POINT ( 'NONE',  ( 39.23433943456829098, -274.3215646882962915, -268.3316149920015619 ) ) ;
#51770=CARTESIAN_POINT ( 'NONE',  ( -6.605048963356055403, -276.1669382116546103, -340.9075191628697326 ) ) ;
#51771=CARTESIAN_POINT ( 'NONE',  ( 96.00430790048001484, -298.2308315540366266, -196.7031297424393586 ) ) ;
#51772=CARTESIAN_POINT ( 'NONE',  ( 26.42467482652973487, -274.2056338440190757, -308.3705234474269332 ) ) ;
#51774=CARTESIAN_POINT ( 'NONE',  ( -34.04045928965716428, -275.1743224558018710, -197.1263729284439989 ) ) ;
#51775=CARTESIAN_POINT ( 'NONE',  ( -24.56713583653360899, -275.1603083401777781, -198.1968209710419444 ) ) ;
#51776=CARTESIAN_POINT ( 'NONE',  ( -35.86813203185662502, -299.6704306543792882, -194.1607190958659714 ) ) ;
#51777=CARTESIAN_POINT ( 'NONE',  ( 24.80271614868557606, -272.9972813898556865, -227.7180730713507160 ) ) ;
#51778=CARTESIAN_POINT ( 'NONE',  ( -92.26178022449579430, -296.5157983408155928, -318.6071278755809431 ) ) ;
#51779=CARTESIAN_POINT ( 'NONE',  ( 20.97916625190972795, -292.7536754211492962, -315.2599282628933679 ) ) ;
#51781=CARTESIAN_POINT ( 'NONE',  ( 20.77788441106363848, -276.7264826566882334, -320.7957481113962785 ) ) ;
#51782=CARTESIAN_POINT ( 'NONE',  ( -51.56353771953207854, -274.0319735407738335, -198.7080757365475279 ) ) ;
#51783=CARTESIAN_POINT ( 'NONE',  ( -111.0210956306622450, -282.9771035354178252, -290.9680331296258942 ) ) ;
#51784=CARTESIAN_POINT ( 'NONE',  ( -112.1167892953612153, -298.4541466750958989, -278.0236544501690332 ) ) ;
#51786=CARTESIAN_POINT ( 'NONE',  ( -70.04545606454857420, -284.8071136175269658, -204.9020058818749419 ) ) ;
#51787=CARTESIAN_POINT ( 'NONE',  ( -111.4060476780554438, -276.7886409042052946, -270.6195273407540185 ) ) ;
#51788=CARTESIAN_POINT ( 'NONE',  ( -81.18486162104123594, -276.2360711649095606, -329.4640122081586924 ) ) ;
#51789=CARTESIAN_POINT ( 'NONE',  ( 18.55066038899585834, -284.2488858665664111, -320.3906144081263392 ) ) ;
#51790=CARTESIAN_POINT ( 'NONE',  ( 35.98277186567027286, -276.7013367957666219, -266.1007085542030381 ) ) ;
#51792=CARTESIAN_POINT ( 'NONE',  ( 38.58166099535635141, -274.0340083866285568, -276.8483091883569500 ) ) ;
#51793=CARTESIAN_POINT ( 'NONE',  ( -3.245082127908186731, -282.5014870486801328, -203.3583181042076831 ) ) ;
#51795=CARTESIAN_POINT ( 'NONE',  ( -18.56397944953064183, -288.2121940331755354, -197.1174924024900577 ) ) ;
#51797=CARTESIAN_POINT ( 'NONE',  ( -89.73759162597615102, -289.3133199411504961, -216.6269217376771508 ) ) ;
#51798=CARTESIAN_POINT ( 'NONE',  ( 82.12584444479689694, -301.3619252513798301, -196.2136339012648421 ) ) ;
#51799=CARTESIAN_POINT ( 'NONE',  ( -77.71767044612955999, -296.2919463044487429, -209.0064025358645665 ) ) ;
#51800=CARTESIAN_POINT ( 'NONE',  ( -105.8337094111578267, -289.0709820956251974, -241.5968699754999420 ) ) ;
#51801=CARTESIAN_POINT ( 'NONE',  ( 26.40820234725076787, -24.66803830325296687, -341.1985388896944755 ) ) ;
#51803=CARTESIAN_POINT ( 'NONE',  ( 11.95305454682809554, -286.8611114333259025, -328.6083060046808555 ) ) ;
#51804=CARTESIAN_POINT ( 'NONE',  ( -26.60648544987661523, -284.5135909336848385, -343.4280182904995513 ) ) ;
#51805=CARTESIAN_POINT ( 'NONE',  ( -113.1392416281361903, -282.8687443791885698, -264.3063662864773278 ) ) ;
#51806=CARTESIAN_POINT ( 'NONE',  ( -109.1789178478847333, -290.3809580755313391, -283.3385657392481676 ) ) ;
#51807=CARTESIAN_POINT ( 'NONE',  ( 35.72708396225598904, -283.0972007792462364, -279.5136551379666798 ) ) ;
#51808=CARTESIAN_POINT ( 'NONE',  ( -18.68461158030488178, -283.6086411758013242, -341.1562353184132235 ) ) ;
#51809=CARTESIAN_POINT ( 'NONE',  ( -107.2626943707492728, -292.1676624055533011, -298.4584730987802459 ) ) ;
#51811=CARTESIAN_POINT ( 'NONE',  ( 4.848023476581549751, -274.9382285887120361, -205.9102099542536735 ) ) ;
#51813=CARTESIAN_POINT ( 'NONE',  ( 32.69816433407451228, -286.0003991606355385, -298.8505309983199254 ) ) ;
#51814=CARTESIAN_POINT ( 'NONE',  ( 2.418001196179785595, -274.5695963131491339, -204.4204920331079052 ) ) ;
#51815=CARTESIAN_POINT ( 'NONE',  ( -4.802211893568830270, -296.6013840662571397, -337.5543205120396237 ) ) ;
#51817=CARTESIAN_POINT ( 'NONE',  ( -85.33152481854864391, -299.9090924074131408, -210.2361428286349110 ) ) ;
#51818=CARTESIAN_POINT ( 'NONE',  ( -8.314775077069059606, -281.3487446853740153, -337.8791237368803309 ) ) ;
#51820=CARTESIAN_POINT ( 'NONE',  ( -108.0217867114887866, -276.2192798760343067, -296.0938644756075746 ) ) ;
#51821=CARTESIAN_POINT ( 'NONE',  ( -65.94916478938755233, -272.1644697477332784, -199.6058535279562705 ) ) ;
#51822=CARTESIAN_POINT ( 'NONE',  ( 33.93500357570439974, -274.6862255737179339, -254.0716954391058948 ) ) ;
#51823=CARTESIAN_POINT ( 'NONE',  ( -22.62087217350328316, -293.7641427854604217, -198.1530507401843124 ) ) ;
#51824=CARTESIAN_POINT ( 'NONE',  ( 24.63274801200521935, -295.0318049131648763, -309.4766047352536020 ) ) ;
#51825=CARTESIAN_POINT ( 'NONE',  ( -111.4042624983455170, -286.3047787658018137, -270.9392790060217635 ) ) ;
#51826=CARTESIAN_POINT ( 'NONE',  ( 36.50838846416730377, -294.7293692528860447, -250.6951106122827753 ) ) ;
#51827=CARTESIAN_POINT ( 'NONE',  ( 37.83751610972370116, -294.6886994617340179, -256.1701448061610336 ) ) ;
#51828=CARTESIAN_POINT ( 'NONE',  ( -68.51926662613033159, -295.3068697202317594, -336.3821168181235635 ) ) ;
#51829=CARTESIAN_POINT ( 'NONE',  ( -110.6112468135569742, -292.3459322671900509, -286.4386582921183617 ) ) ;
#51830=CARTESIAN_POINT ( 'NONE',  ( -101.4179626534740635, -284.1557502113835767, -313.1561121816219497 ) ) ;
#51831=CARTESIAN_POINT ( 'NONE',  ( -35.49079075278447704, -296.1550023229804083, -194.8017099911895684 ) ) ;
#51832=CARTESIAN_POINT ( 'NONE',  ( -112.5255515072295935, -284.1775553355857937, -286.9860539624092439 ) ) ;
#51833=CARTESIAN_POINT ( 'NONE',  ( -105.7693302352541735, -280.1383373422133900, -300.3151256840215524 ) ) ;
#51834=CARTESIAN_POINT ( 'NONE',  ( -109.8107469201079169, -283.5007667540454008, -258.6468452431744254 ) ) ;
#51835=CARTESIAN_POINT ( 'NONE',  ( 33.95594074649907412, -285.2494619234425954, -246.9215409384524378 ) ) ;
#51836=CARTESIAN_POINT ( 'NONE',  ( -110.5315628778188994, -276.9415308877714210, -250.7266713465869259 ) ) ;
#51837=CARTESIAN_POINT ( 'NONE',  ( -112.8392349625790274, -266.9846182459017427, -270.2902299390011081 ) ) ;
#51838=CARTESIAN_POINT ( 'NONE',  ( -94.16595011483481414, -284.7089361065579283, -224.4175175083425415 ) ) ;
#51839=CARTESIAN_POINT ( 'NONE',  ( 33.94922476129675459, -282.3984064311338784, -242.1876307228529868 ) ) ;
#51840=CARTESIAN_POINT ( 'NONE',  ( -62.69728083778057481, -288.4328759412251770, -342.8736287742139552 ) ) ;
#51841=CARTESIAN_POINT ( 'NONE',  ( -96.42107494180385174, -279.4994528838173551, -318.5070877323978493 ) ) ;
#51842=CARTESIAN_POINT ( 'NONE',  ( 10.23258619427804206, -277.7270409929954553, -330.3452673534020505 ) ) ;
#51843=CARTESIAN_POINT ( 'NONE',  ( -76.82007195183167880, -279.3409834169878536, -208.8968036737456373 ) ) ;
#51844=CARTESIAN_POINT ( 'NONE',  ( 8.317561934251690658, -276.6604562315231419, -211.3096269979002386 ) ) ;
#51845=CARTESIAN_POINT ( 'NONE',  ( 38.06190843432031556, -293.3562701668817567, -254.6985520459939494 ) ) ;
#51846=CARTESIAN_POINT ( 'NONE',  ( 20.95915198056814077, -284.9047667132333572, -223.4255745101119714 ) ) ;
#51848=CARTESIAN_POINT ( 'NONE',  ( -36.40884667172176847, -293.6637864842886643, -194.1539289451806667 ) ) ;
#51850=CARTESIAN_POINT ( 'NONE',  ( 1.722969254557689123, -293.4369771981951658, -332.4549142219471491 ) ) ;
#51851=CARTESIAN_POINT ( 'NONE',  ( 19.70762346661165410, -293.8627343345103782, -315.9602349079602277 ) ) ;
#51853=CARTESIAN_POINT ( 'NONE',  ( -112.5621054832894998, -291.4433097802354951, -285.3736299110723280 ) ) ;
#51854=CARTESIAN_POINT ( 'NONE',  ( -1.923946207189996205, -281.1859637584270786, -206.4121119265851121 ) ) ;
#51855=CARTESIAN_POINT ( 'NONE',  ( -76.30293345726610710, -272.6037346133413735, -204.1571100663524589 ) ) ;
#51856=CARTESIAN_POINT ( 'NONE',  ( 23.21233099692946666, -288.8381278299563064, -317.7798135117720335 ) ) ;
#51857=CARTESIAN_POINT ( 'NONE',  ( 22.41386763608326405, -280.3244136636627672, -316.9608001777151003 ) ) ;
#51858=CARTESIAN_POINT ( 'NONE',  ( -3.066332952619674312, -288.9450693959109344, -339.3028311170559732 ) ) ;
#51859=CARTESIAN_POINT ( 'NONE',  ( -30.53353787668844177, -286.4737532708497270, -197.6072347239738178 ) ) ;
#51860=CARTESIAN_POINT ( 'NONE',  ( 84.21812867672285563, 83.45443861182893386, -302.1763853415790209 ) ) ;
#51861=CARTESIAN_POINT ( 'NONE',  ( -84.98320358907332661, -218.2615186942531409, -350.7060260155240030 ) ) ;
#51862=CARTESIAN_POINT ( 'NONE',  ( 173.1604602154851875, 240.6435161624839338, -177.0232263525105907 ) ) ;
#51863=CARTESIAN_POINT ( 'NONE',  ( -72.19765763824351268, -278.7756547176378490, -206.0364418984405006 ) ) ;
#51864=CARTESIAN_POINT ( 'NONE',  ( -108.1222861304432854, -277.2214165994359405, -289.4486720284914441 ) ) ;
#51865=CARTESIAN_POINT ( 'NONE',  ( -114.3203984661416399, -272.2547862396379514, -267.4902059702777706 ) ) ;
#51866=CARTESIAN_POINT ( 'NONE',  ( 26.98300397726301725, -24.65525921013767885, -342.2912574563407020 ) ) ;
#51867=ADVANCED_FACE ( 'NONE', ( #93300 ), #28450, .T. ) ;
#51868=CARTESIAN_POINT ( 'NONE',  ( -19.87315442162139334, -278.8470366021491600, -195.9195587694034941 ) ) ;
#51869=CARTESIAN_POINT ( 'NONE',  ( -14.07078513763565297, -296.5144743677850556, -342.6967145281109310 ) ) ;
#51870=CARTESIAN_POINT ( 'NONE',  ( -79.57138049760347087, -291.9569396937159240, -210.6782799074938737 ) ) ;
#51871=CARTESIAN_POINT ( 'NONE',  ( -76.32360360301103697, -274.4859349289054649, -204.1692798212957314 ) ) ;
#51872=CARTESIAN_POINT ( 'NONE',  ( -10.55989518150903983, -287.3802701280101815, -338.8552912570969511 ) ) ;
#51873=CARTESIAN_POINT ( 'NONE',  ( -102.6368702000801676, -273.7356421530424200, -229.7427286533957442 ) ) ;
#51874=CARTESIAN_POINT ( 'NONE',  ( -109.2762201800415340, -296.8827627635618001, -257.9343392603321945 ) ) ;
#51878=CARTESIAN_POINT ( 'NONE',  ( -94.82649853260295458, -281.1464848322396506, -221.3023529691275542 ) ) ;
#51881=CARTESIAN_POINT ( 'NONE',  ( -110.2751131314128799, -279.7356011958916042, -262.4613132416062626 ) ) ;
#51882=CARTESIAN_POINT ( 'NONE',  ( -113.3706383089800056, -280.2964112198901034, -271.6143522394123693 ) ) ;
#51883=CARTESIAN_POINT ( 'NONE',  ( -67.32201083455039736, -272.1315862647464883, -203.0279926872035219 ) ) ;
#51886=CARTESIAN_POINT ( 'NONE',  ( -68.52521708756100338, -279.7972491266701809, -204.3566615074421691 ) ) ;
#51888=CARTESIAN_POINT ( 'NONE',  ( 35.05228750150188688, -276.6824700767942886, -296.2720261306258749 ) ) ;
#51889=CARTESIAN_POINT ( 'NONE',  ( 28.79185429016951048, -278.0229503667779909, -305.8453205207046040 ) ) ;
#51890=CARTESIAN_POINT ( 'NONE',  ( -37.14683262218385806, -275.6244569760258400, -346.7846013406943371 ) ) ;
#51893=CARTESIAN_POINT ( 'NONE',  ( 32.06111909379272618, -283.9153081272322083, -299.8484504907859218 ) ) ;
#51894=CARTESIAN_POINT ( 'NONE',  ( -102.5488586488664993, -290.2002487404811859, -237.0732866943937154 ) ) ;
#51895=CARTESIAN_POINT ( 'NONE',  ( -46.48513868308838681, -285.2875884870334176, -194.0085782880030933 ) ) ;
#51896=CARTESIAN_POINT ( 'NONE',  ( -101.2877509435486587, -282.2875545616817021, -307.6287526927116005 ) ) ;
#51897=CARTESIAN_POINT ( 'NONE',  ( -38.91573687095960565, -281.6469709578629477, -343.9461045972946067 ) ) ;
#51898=CARTESIAN_POINT ( 'NONE',  ( 28.95146729627809634, -285.1795373793448789, -236.3869425068192527 ) ) ;
#51899=CARTESIAN_POINT ( 'NONE',  ( -27.52035372606641772, -281.3846391851541853, -197.5726463987835189 ) ) ;
#51900=CARTESIAN_POINT ( 'NONE',  ( 180.5981353652897496, 255.9489591101111046, -166.9704198444101451 ) ) ;
#51901=CARTESIAN_POINT ( 'NONE',  ( 10.96949821822724935, -280.7966828342952113, -329.3570384045843298 ) ) ;
#51902=CARTESIAN_POINT ( 'NONE',  ( 35.47391973830447398, -295.3215238129108116, -252.3920847284757940 ) ) ;
#51904=CARTESIAN_POINT ( 'NONE',  ( -109.5915464334587881, -279.0569643513442202, -281.4900162715477450 ) ) ;
#51905=CARTESIAN_POINT ( 'NONE',  ( -54.56975096601541964, -287.8314300844096465, -197.1953972673855162 ) ) ;
#51907=CARTESIAN_POINT ( 'NONE',  ( -96.35454364961768192, -293.1163991317904447, -223.1721520866158812 ) ) ;
#51909=CARTESIAN_POINT ( 'NONE',  ( -21.24802395708481839, -274.8456881303112596, -343.6674775021141386 ) ) ;
#51910=CARTESIAN_POINT ( 'NONE',  ( 30.21583466696752751, -287.2251493141621381, -307.0802679876832713 ) ) ;
#51911=CARTESIAN_POINT ( 'NONE',  ( 35.62584744216544408, -292.1005805504409523, -281.7463104529301177 ) ) ;
#51912=CARTESIAN_POINT ( 'NONE',  ( -68.26003287896597271, -276.1517906428187530, -337.0480445774149985 ) ) ;
#51913=CARTESIAN_POINT ( 'NONE',  ( -109.8026360077661110, -294.4824546312578377, -286.4942595045956182 ) ) ;
#51914=CARTESIAN_POINT ( 'NONE',  ( -70.17783218354340136, -290.8093332610928883, -336.1248361181010864 ) ) ;
#51917=CARTESIAN_POINT ( 'NONE',  ( 20.79489701036722238, -291.3594542414228385, -220.9160160474684744 ) ) ;
#51918=CARTESIAN_POINT ( 'NONE',  ( -7.954914001910267096, -288.0438491317030980, -202.6643143814241341 ) ) ;
#51919=CARTESIAN_POINT ( 'NONE',  ( -110.6491946599201839, -289.0464139752578490, -250.3121678261010459 ) ) ;
#51920=CARTESIAN_POINT ( 'NONE',  ( -3.075960133487551929, -290.0157804865847879, -335.5423201903118411 ) ) ;
#51922=CARTESIAN_POINT ( 'NONE',  ( -31.84905003557559411, -289.7840476326607018, -343.3668567379307319 ) ) ;
#51923=CARTESIAN_POINT ( 'NONE',  ( -78.55583616408829073, -297.5840318635425206, -333.4467882404397301 ) ) ;
#51925=CARTESIAN_POINT ( 'NONE',  ( 33.67998897336980946, -289.1251258290616875, -299.2066293557593326 ) ) ;
#51926=CARTESIAN_POINT ( 'NONE',  ( -108.9780180173413981, -276.8747278547912174, -246.8152435183763771 ) ) ;
#51927=CARTESIAN_POINT ( 'NONE',  ( -45.27541442975697095, -280.2876777570410809, -193.7392158406236717 ) ) ;
#51928=CARTESIAN_POINT ( 'NONE',  ( -67.35030184351538196, -279.3359297978559539, -199.4722746103293787 ) ) ;
#51929=CARTESIAN_POINT ( 'NONE',  ( -65.82993802584303467, -283.6794743266306682, -200.9270235732126650 ) ) ;
#51931=CARTESIAN_POINT ( 'NONE',  ( -39.71742228385635798, -278.1616160560209323, -196.1512067622547306 ) ) ;
#51932=CARTESIAN_POINT ( 'NONE',  ( -98.18143222490674304, -281.9539909847155172, -314.3059858516032818 ) ) ;
#51934=CARTESIAN_POINT ( 'NONE',  ( -111.4082183218339424, -277.2643426227267014, -251.9538567227673695 ) ) ;
#51935=CARTESIAN_POINT ( 'NONE',  ( 9.462241287838949688, -300.1685837963163408, -196.6554053896869618 ) ) ;
#51936=CARTESIAN_POINT ( 'NONE',  ( -90.23494134184763027, -282.6992769371827308, -325.9658973063937424 ) ) ;
#51937=CARTESIAN_POINT ( 'NONE',  ( -64.63850758792814588, -274.4892669104845027, -202.4691422519154003 ) ) ;
#51938=CARTESIAN_POINT ( 'NONE',  ( -103.7266816256837814, -274.4738267847678230, -232.4178644756300969 ) ) ;
#51939=CARTESIAN_POINT ( 'NONE',  ( 35.60834090647416161, -275.1632275029686525, -266.1419785265910036 ) ) ;
#51940=CARTESIAN_POINT ( 'NONE',  ( -35.57874820471536026, -297.0302193861775208, -345.3532376387585714 ) ) ;
#51941=CARTESIAN_POINT ( 'NONE',  ( -98.15830030560384500, -290.0881284591212648, -317.5876057556349110 ) ) ;
#51942=CARTESIAN_POINT ( 'NONE',  ( -56.17367249863987411, -277.8913964011774169, -197.1315337419543994 ) ) ;
#51943=CARTESIAN_POINT ( 'NONE',  ( -108.3663174189062346, -290.7637549701123589, -240.6205103361294562 ) ) ;
#51944=CARTESIAN_POINT ( 'NONE',  ( -88.83499678121414433, -288.8561930924760759, -322.4365329848433817 ) ) ;
#51945=CARTESIAN_POINT ( 'NONE',  ( 35.15657629717884447, -291.7988961774175323, -289.5705054500083975 ) ) ;
#51949=CARTESIAN_POINT ( 'NONE',  ( -99.76093133645639455, -290.5823294157507348, -232.3897074618980128 ) ) ;
#51951=CARTESIAN_POINT ( 'NONE',  ( 16.12668598135667608, -287.7298505218980154, -215.2797971977761620 ) ) ;
#51952=CARTESIAN_POINT ( 'NONE',  ( 27.36219212280431989, -296.4805209788416391, -301.4846348637938149 ) ) ;
#51953=CARTESIAN_POINT ( 'NONE',  ( -32.04076049171884932, -294.0455973034375461, -346.9557935645869406 ) ) ;
#51954=CARTESIAN_POINT ( 'NONE',  ( -1.847961186025400826, -283.9070645179809844, -338.1364288995113156 ) ) ;
#51955=CARTESIAN_POINT ( 'NONE',  ( -73.55378684275576973, -285.3905892891570488, -206.9614126473610156 ) ) ;
#51957=CARTESIAN_POINT ( 'NONE',  ( 35.32677200703673748, -276.7223648358997821, -259.2976522769824328 ) ) ;
#51958=CARTESIAN_POINT ( 'NONE',  ( 15.46238967421055044, -292.3217590176546992, -323.1933628464565231 ) ) ;
#51959=CARTESIAN_POINT ( 'NONE',  ( 13.78418317186730668, -273.5835759955461981, -217.6992289062438886 ) ) ;
#51962=CARTESIAN_POINT ( 'NONE',  ( -11.06841617541174472, -294.3857287583105631, -342.7741411782204750 ) ) ;
#51963=CARTESIAN_POINT ( 'NONE',  ( 24.72137977662807273, -288.9119320753017064, -229.1644530640811581 ) ) ;
#51964=CARTESIAN_POINT ( 'NONE',  ( -109.1432659898178059, -297.2879090788925396, -297.4557723210269842 ) ) ;
#51966=CARTESIAN_POINT ( 'NONE',  ( 22.06958145142643701, -287.6080311963875147, -227.6824515807841465 ) ) ;
#51968=CARTESIAN_POINT ( 'NONE',  ( -100.2794831484175404, -277.0281520501196724, -314.3117230024359969 ) ) ;
#51969=CARTESIAN_POINT ( 'NONE',  ( 39.60961157373269970, -294.2028207387753014, -270.3017462191357367 ) ) ;
#51970=CARTESIAN_POINT ( 'NONE',  ( 29.26531416745986647, -286.1677361792641250, -306.5791032641260472 ) ) ;
#51971=CARTESIAN_POINT ( 'NONE',  ( 36.26551863187449243, -293.6024214982456897, -247.8284386489340818 ) ) ;
#51972=CARTESIAN_POINT ( 'NONE',  ( -79.54638421528115089, -291.7978992803895721, -210.7101114339929779 ) ) ;
#51975=CARTESIAN_POINT ( 'NONE',  ( -112.3417001281054723, -270.5523139186827279, -270.3356821209761165 ) ) ;
#51976=CARTESIAN_POINT ( 'NONE',  ( 139.1551670580431619, 178.0905500625548257, -238.3682463250823389 ) ) ;
#51977=CARTESIAN_POINT ( 'NONE',  ( 38.94646215847269133, -289.0510653369147462, -268.6806282160406454 ) ) ;
#51978=CARTESIAN_POINT ( 'NONE',  ( 13.84574458161073807, -290.1952119285918457, -206.2264541496106460 ) ) ;
#51980=CARTESIAN_POINT ( 'NONE',  ( -10.87695737206971103, -281.6192572698207641, -338.7804342335923593 ) ) ;
#51981=CARTESIAN_POINT ( 'NONE',  ( -97.91489887575750117, -277.5836653927943871, -317.8651376559970458 ) ) ;
#51982=CARTESIAN_POINT ( 'NONE',  ( 1.325988064423260893, -282.5696769496167917, -206.2321321975770729 ) ) ;
#51983=CARTESIAN_POINT ( 'NONE',  ( -111.0079197358586214, -274.0791632895269458, -270.3805604919635925 ) ) ;
#51984=CARTESIAN_POINT ( 'NONE',  ( -52.04200835963407457, -284.4424090379778249, -195.3237669500531979 ) ) ;
#51985=CARTESIAN_POINT ( 'NONE',  ( 31.48800536491854629, -285.1916654029594724, -241.3425825247887531 ) ) ;
#51986=CARTESIAN_POINT ( 'NONE',  ( -3.136734348080123524, -276.3594654734198457, -202.7424681462508715 ) ) ;
#51988=CARTESIAN_POINT ( 'NONE',  ( -90.09463718365785212, -297.7740240719996905, -219.7405530229252406 ) ) ;
#51990=CARTESIAN_POINT ( 'NONE',  ( 18.33514920658155489, -292.9158128532565115, -318.3525001728627899 ) ) ;
#51991=CARTESIAN_POINT ( 'NONE',  ( -112.3831137694602091, -278.9932285075610707, -287.1569218002958905 ) ) ;
#51992=CARTESIAN_POINT ( 'NONE',  ( -61.78982515148061339, -277.3787944179788383, -339.1992259225982593 ) ) ;
#51993=CARTESIAN_POINT ( 'NONE',  ( -9.229482989995716480, -299.3372925595347169, -193.5920387966222620 ) ) ;
#51994=CARTESIAN_POINT ( 'NONE',  ( -100.2199783508677911, -276.8897549883956799, -314.2680039770266376 ) ) ;
#51995=CARTESIAN_POINT ( 'NONE',  ( 189.2871950347156940, 271.4890288425742142, -139.5295763810835865 ) ) ;
#51996=CARTESIAN_POINT ( 'NONE',  ( 34.98873975703526185, -273.8075871038321338, -290.2410010562821299 ) ) ;
#51998=CARTESIAN_POINT ( 'NONE',  ( -92.26079611022613847, -297.2439526662178650, -323.4883161862781549 ) ) ;
#51999=CARTESIAN_POINT ( 'NONE',  ( -85.33152481854864391, -275.9090924074130839, -210.2361428286349110 ) ) ;
#52000=CARTESIAN_POINT ( 'NONE',  ( -30.04969936926732288, -125.9919632799748683, -361.3284013991797110 ) ) ;
#52001=CARTESIAN_POINT ( 'NONE',  ( -109.7285362384405119, -285.7851450106398943, -258.6896161597846913 ) ) ;
#52002=CARTESIAN_POINT ( 'NONE',  ( -89.72315216868167909, -285.5386321713770599, -325.4801096333073929 ) ) ;
#52003=CARTESIAN_POINT ( 'NONE',  ( -57.41442229614335702, -285.1348590589498144, -200.0163390994463271 ) ) ;
#52004=CARTESIAN_POINT ( 'NONE',  ( -89.66725952945785139, -276.2046951007795315, -322.4767296067391271 ) ) ;
#52005=CARTESIAN_POINT ( 'NONE',  ( -102.0799160549964881, -286.9026059667446020, -233.9262625125008981 ) ) ;
#52006=CARTESIAN_POINT ( 'NONE',  ( -59.92789630099822773, -278.2341207688878058, -200.1605263892135724 ) ) ;
#52007=CARTESIAN_POINT ( 'NONE',  ( 27.04479631321792610, -277.1095257163754013, -305.5187383069378484 ) ) ;
#52009=CARTESIAN_POINT ( 'NONE',  ( -97.89770967483167396, -273.6132652578792204, -229.3934956482949588 ) ) ;
#52010=CARTESIAN_POINT ( 'NONE',  ( 34.17038043787031398, -281.9962280459111525, -242.1057839266462395 ) ) ;
#52011=CARTESIAN_POINT ( 'NONE',  ( -30.21434691575735343, -283.4566042545496884, -346.9687399230846836 ) ) ;
#52016=CARTESIAN_POINT ( 'NONE',  ( -21.26946536258823528, -288.1166067479214234, -196.3206645302480524 ) ) ;
#52017=CARTESIAN_POINT ( 'NONE',  ( -110.3165667304556479, -288.9444064529691332, -293.5118513105415445 ) ) ;
#52018=CARTESIAN_POINT ( 'NONE',  ( -110.5355835966617519, -295.7709277141003099, -268.7190931944208501 ) ) ;
#52019=CARTESIAN_POINT ( 'NONE',  ( 13.21770259551357007, -292.0862236448231783, -212.4209800596536297 ) ) ;
#52020=CARTESIAN_POINT ( 'NONE',  ( 1.662291437309062703, -287.0001007713279932, -332.8862840670425385 ) ) ;
#52021=CARTESIAN_POINT ( 'NONE',  ( 14.48559661566718049, -286.8800168204973033, -322.6038804362329984 ) ) ;
#52022=CARTESIAN_POINT ( 'NONE',  ( -36.16788276254150247, -290.3068895503973295, -196.3444405872138248 ) ) ;
#52023=CARTESIAN_POINT ( 'NONE',  ( -68.95981749745881473, -286.8319300749523109, -204.1096102392688749 ) ) ;
#52024=CARTESIAN_POINT ( 'NONE',  ( -109.4082310404863279, -276.8193602355277108, -249.5905673760453851 ) ) ;
#52025=CARTESIAN_POINT ( 'NONE',  ( 28.20510820910030958, -286.4636447299458837, -309.2205612473138672 ) ) ;
#52027=CARTESIAN_POINT ( 'NONE',  ( -20.90913801687735685, -290.8415605589049164, -343.5920408286086172 ) ) ;
#52028=CARTESIAN_POINT ( 'NONE',  ( -90.32477883102639282, -287.7990660290804499, -323.7524817515514428 ) ) ;
#52029=CARTESIAN_POINT ( 'NONE',  ( -7.145544870866885390, -283.5872817200231566, -337.0951936600899330 ) ) ;
#52030=CARTESIAN_POINT ( 'NONE',  ( -78.60968204390852065, -293.4984325607915139, -207.4738745102226858 ) ) ;
#52034=CARTESIAN_POINT ( 'NONE',  ( -57.03836387379394068, -299.7203185958575773, -197.3592459473535996 ) ) ;
#52035=CARTESIAN_POINT ( 'NONE',  ( 30.17443138965062133, -280.3721281583601126, -242.1800301505892890 ) ) ;
#52036=CARTESIAN_POINT ( 'NONE',  ( 22.11668210822592329, -278.9256080486096039, -224.6269826264428104 ) ) ;
#52037=CARTESIAN_POINT ( 'NONE',  ( 36.21212761405281810, -293.0309283784445711, -292.7672370760836884 ) ) ;
#52038=CARTESIAN_POINT ( 'NONE',  ( -100.1284166468338981, -271.3255263694940140, -231.1718051364767632 ) ) ;
#52039=CARTESIAN_POINT ( 'NONE',  ( 23.63154270290049652, -274.2170828571468633, -313.1529453722600920 ) ) ;
#52040=CARTESIAN_POINT ( 'NONE',  ( -53.23984682951795833, -296.5753475943707826, -342.1664472209325822 ) ) ;
#52043=CARTESIAN_POINT ( 'NONE',  ( -109.8398071270582079, -294.5017166221026628, -293.1642916526852218 ) ) ;
#52045=CARTESIAN_POINT ( 'NONE',  ( 23.42976964351907299, -295.5512854999624324, -311.9496961033782441 ) ) ;
#52047=CARTESIAN_POINT ( 'NONE',  ( -75.73410897391093499, -296.3813508877580034, -332.6987820336518098 ) ) ;
#52049=CARTESIAN_POINT ( 'NONE',  ( -92.69403831484001444, -283.2843834615023866, -219.1522432961410516 ) ) ;
#52050=CARTESIAN_POINT ( 'NONE',  ( -98.44757094535637520, -297.1067407774778530, -230.3312834648069440 ) ) ;
#52052=CARTESIAN_POINT ( 'NONE',  ( -70.47011812078504533, -283.4768185056325933, -339.8846287775337487 ) ) ;
#52053=CARTESIAN_POINT ( 'NONE',  ( 18.73162842497693958, -284.1737779572890759, -321.0844736798899248 ) ) ;
#52054=CARTESIAN_POINT ( 'NONE',  ( -68.48831159718943695, -285.3207193823188277, -199.9504898604309062 ) ) ;
#52055=CARTESIAN_POINT ( 'NONE',  ( -87.13026657072720127, -289.3570090150861347, -214.4243442208789361 ) ) ;
#52056=CARTESIAN_POINT ( 'NONE',  ( 35.78497577281001440, -272.8380690714490129, -253.7030783399848985 ) ) ;
#52059=CARTESIAN_POINT ( 'NONE',  ( 30.42293856315230371, -285.8562765816720912, -241.7828628820301446 ) ) ;
#52060=CARTESIAN_POINT ( 'NONE',  ( -100.4341511263454265, -288.8944097929862096, -313.9596860432638437 ) ) ;
#52062=CARTESIAN_POINT ( 'NONE',  ( -105.5088612183088799, -298.5273794335520279, -242.0825295758795335 ) ) ;
#52063=CARTESIAN_POINT ( 'NONE',  ( -96.37389219554266617, -280.6343093657642385, -221.8247215083474089 ) ) ;
#52064=CARTESIAN_POINT ( 'NONE',  ( 26.69459508139615522, -292.1042328646184387, -310.1801234095037785 ) ) ;
#52065=CARTESIAN_POINT ( 'NONE',  ( 21.82657927533756492, -281.8175891192346398, -313.1750736549134899 ) ) ;
#52066=CARTESIAN_POINT ( 'NONE',  ( -22.09547090729973107, -295.0286947913670588, -345.8366272490243318 ) ) ;
#52067=CARTESIAN_POINT ( 'NONE',  ( -103.1746369036387705, -282.1404074073567472, -307.5527081642565008 ) ) ;
#52068=CARTESIAN_POINT ( 'NONE',  ( -112.0540594091986293, -280.6438772246250437, -263.2300970651955936 ) ) ;
#52069=CARTESIAN_POINT ( 'NONE',  ( -6.677270644135938404, -293.6981034536681818, -336.8675177743754148 ) ) ;
#52070=CARTESIAN_POINT ( 'NONE',  ( -103.9717408117783322, -271.0130733286139275, -235.4569417527998496 ) ) ;
#52073=CARTESIAN_POINT ( 'NONE',  ( 12.38316218089645027, -282.7286526451247823, -214.6898967956778108 ) ) ;
#52074=CARTESIAN_POINT ( 'NONE',  ( -107.5167301283792369, -296.3285219301502025, -250.0275593611395095 ) ) ;
#52076=CARTESIAN_POINT ( 'NONE',  ( 21.31550574532286291, -272.4094976428775681, -223.6242672951989618 ) ) ;
#52077=CARTESIAN_POINT ( 'NONE',  ( -76.34192880043993057, -272.7421316953116275, -204.0943482722793760 ) ) ;
#52078=CARTESIAN_POINT ( 'NONE',  ( -92.55510678622148646, -291.0659355605029646, -222.6067492847590188 ) ) ;
#52079=CARTESIAN_POINT ( 'NONE',  ( -94.49035528878833645, -280.7246287572394294, -223.8343625843774873 ) ) ;
#52080=CARTESIAN_POINT ( 'NONE',  ( -27.20018825017380237, -275.7831862839449855, -197.2097985232132658 ) ) ;
#52081=CARTESIAN_POINT ( 'NONE',  ( 21.91415590932306046, -283.8015893952864985, -318.2897904512860805 ) ) ;
#52082=CARTESIAN_POINT ( 'NONE',  ( -74.69471913953061915, -278.3383767729300189, -207.1213605377907072 ) ) ;
#52083=CARTESIAN_POINT ( 'NONE',  ( -74.99594713437370785, -279.5539075098164403, -335.2237291813885349 ) ) ;
#52084=ORIENTED_EDGE ( 'NONE', *, *, #37335, .T. ) ;
#52085=CARTESIAN_POINT ( 'NONE',  ( -96.02631077693312989, -273.0576806687402041, -220.4898750584278844 ) ) ;
#52086=CARTESIAN_POINT ( 'NONE',  ( 5.309071489689258350, -294.5539435640115471, -209.2878970248545443 ) ) ;
#52090=CARTESIAN_POINT ( 'NONE',  ( -53.05655803448743058, -293.3909756074681354, -344.5319182710871928 ) ) ;
#52091=CARTESIAN_POINT ( 'NONE',  ( -109.9462226093743311, -272.1673443876977672, -262.2019662576451537 ) ) ;
#52093=CARTESIAN_POINT ( 'NONE',  ( 32.68042373087087782, -294.6823127120879349, -240.0360471453423088 ) ) ;
#52094=CARTESIAN_POINT ( 'NONE',  ( -54.49178911615187815, -276.3376638359844151, -195.3683826091709363 ) ) ;
#52095=CARTESIAN_POINT ( 'NONE',  ( 37.28218010577872121, -289.6327263608534395, -276.6096840821182923 ) ) ;
#52096=CARTESIAN_POINT ( 'NONE',  ( -29.54717560293130774, -274.9531837356862525, -344.8395990932402242 ) ) ;
#52097=CARTESIAN_POINT ( 'NONE',  ( 35.58003269586576778, -277.6658072258828156, -285.3188946530946737 ) ) ;
#52098=CARTESIAN_POINT ( 'NONE',  ( 20.80352015777070207, -292.2761184254233058, -316.8620439614169300 ) ) ;
#52099=CARTESIAN_POINT ( 'NONE',  ( -111.2029559986527261, -280.6270680120944121, -253.4844960936010239 ) ) ;
#52101=CARTESIAN_POINT ( 'NONE',  ( -38.88978253256773598, -282.7387854184567573, -343.3783446526049943 ) ) ;
#52102=CARTESIAN_POINT ( 'NONE',  ( -5.086556778380232124, -281.5465589776422348, -200.7831168718684296 ) ) ;
#52103=CARTESIAN_POINT ( 'NONE',  ( -61.12305409306145521, -282.1489762642081587, -343.2344838265923954 ) ) ;
#52104=CARTESIAN_POINT ( 'NONE',  ( -71.45548342034609846, -278.4329685435018291, -339.1293519536326357 ) ) ;
#52107=CARTESIAN_POINT ( 'NONE',  ( 36.57202372075288821, -277.3116924913637718, -289.3207904847089935 ) ) ;
#52108=CARTESIAN_POINT ( 'NONE',  ( 7.450504543161046378, -290.9090924074130839, -326.4764044574609443 ) ) ;
#52110=CARTESIAN_POINT ( 'NONE',  ( -108.7663181958378402, -298.2550165232029826, -293.4097201547684790 ) ) ;
#52111=CARTESIAN_POINT ( 'NONE',  ( -66.70043993297734630, -292.7379041519777161, -203.1875333574132583 ) ) ;
#52112=CARTESIAN_POINT ( 'NONE',  ( -54.35273317160154249, -275.2916962491779600, -343.0950508506979872 ) ) ;
#52113=CARTESIAN_POINT ( 'NONE',  ( -3.491738771969169264, -290.3716985335921663, -338.4060939883290757 ) ) ;
#52114=CARTESIAN_POINT ( 'NONE',  ( -0.03180194821504418734, -291.9115320143268946, -207.4972637735380374 ) ) ;
#52115=CARTESIAN_POINT ( 'NONE',  ( -17.74605439000924889, -288.3136220129707681, -344.7623113276230242 ) ) ;
#52117=CARTESIAN_POINT ( 'NONE',  ( -109.4421566815660185, -283.1582669041812892, -254.5553008887981719 ) ) ;
#52118=CARTESIAN_POINT ( 'NONE',  ( -107.1868467685962116, -292.0831787502150974, -295.5110875619837429 ) ) ;
#52119=CARTESIAN_POINT ( 'NONE',  ( -101.0097886998090786, -282.5275351611591645, -307.4701768336705641 ) ) ;
#52120=CARTESIAN_POINT ( 'NONE',  ( 34.23691015205043442, -282.6489508754667668, -253.6954037747211714 ) ) ;
#52121=CARTESIAN_POINT ( 'NONE',  ( -97.09933241152299388, -290.8452386798986709, -318.5673772053381185 ) ) ;
#52122=CARTESIAN_POINT ( 'NONE',  ( -101.9083808232471284, -278.5791308149198926, -304.5536929876997760 ) ) ;
#52123=CARTESIAN_POINT ( 'NONE',  ( 10.88079596109349723, -291.4968410130016991, -210.7731203460172651 ) ) ;
#52125=CARTESIAN_POINT ( 'NONE',  ( -1.054859161684753355, -287.3241470186201241, -202.6305931543492704 ) ) ;
#52126=CARTESIAN_POINT ( 'NONE',  ( 19.58294209324710522, -288.7486735338324593, -322.1408827900740448 ) ) ;
#52127=CARTESIAN_POINT ( 'NONE',  ( -83.64950768871226217, -285.5630604454160562, -213.8632928156920343 ) ) ;
#52130=CARTESIAN_POINT ( 'NONE',  ( 36.84748508202453365, -295.2163851412431086, -254.9265398853929980 ) ) ;
#52131=CARTESIAN_POINT ( 'NONE',  ( -106.7262191213813622, -294.8217780197038564, -302.5959872314968493 ) ) ;
#52133=CARTESIAN_POINT ( 'NONE',  ( -54.01912345500431201, -276.3301693208909455, -341.7245218092296000 ) ) ;
#52134=CARTESIAN_POINT ( 'NONE',  ( -100.6620113337510674, -296.4778262537071214, -226.7048401822121946 ) ) ;
#52135=CARTESIAN_POINT ( 'NONE',  ( 21.87213777095738720, -292.6413495833809861, -314.2294340561453510 ) ) ;
#52136=CARTESIAN_POINT ( 'NONE',  ( -72.12162973394761423, -295.8254644295049047, -205.0142636252858779 ) ) ;
#52137=CARTESIAN_POINT ( 'NONE',  ( -49.77098528653240095, -293.0953032023202240, -197.9724993497362391 ) ) ;
#52138=CARTESIAN_POINT ( 'NONE',  ( 20.41797872154405979, -293.9979210339787414, -225.1960817692392425 ) ) ;
#52140=CARTESIAN_POINT ( 'NONE',  ( 33.74409460231963465, -291.8692495823948434, -294.9507337451625517 ) ) ;
#52141=CARTESIAN_POINT ( 'NONE',  ( -95.90639019058509973, -297.9078327160810886, -317.2339742737384540 ) ) ;
#52142=CARTESIAN_POINT ( 'NONE',  ( -99.03353974879111377, -290.9492539205385242, -309.8266139531350518 ) ) ;
#52143=CARTESIAN_POINT ( 'NONE',  ( -68.52251281566290686, -295.8067499217232807, -336.4039708155657991 ) ) ;
#52144=CARTESIAN_POINT ( 'NONE',  ( -98.91977470617750612, -281.1192740225314992, -226.9267130101486885 ) ) ;
#52145=CARTESIAN_POINT ( 'NONE',  ( -86.47511438163938635, -278.0713825403471446, -211.6473367878045906 ) ) ;
#52146=CARTESIAN_POINT ( 'NONE',  ( -81.18545255908168201, -272.8223834378584343, -207.1219326708940400 ) ) ;
#52147=CARTESIAN_POINT ( 'NONE',  ( 8.665118925045300458, -280.4963604258299483, -328.9477567559068234 ) ) ;
#52148=CARTESIAN_POINT ( 'NONE',  ( -79.45153693740967071, -277.8940040383092764, -206.7903372285142893 ) ) ;
#52149=CARTESIAN_POINT ( 'NONE',  ( -39.16387900916373610, -296.7136680926682288, -196.8780653055216590 ) ) ;
#52152=CARTESIAN_POINT ( 'NONE',  ( -111.2596184192468343, -288.3842409438140066, -285.0740933994331954 ) ) ;
#52153=CARTESIAN_POINT ( 'NONE',  ( -70.63907033646067646, -289.4791001695629689, -339.8038771182556843 ) ) ;
#52154=CARTESIAN_POINT ( 'NONE',  ( -70.61474256897695057, -275.6145636512155193, -202.9598340352300454 ) ) ;
#52155=CARTESIAN_POINT ( 'NONE',  ( -111.5581852811192931, -270.6953707836397029, -259.1943451678488941 ) ) ;
#52156=CARTESIAN_POINT ( 'NONE',  ( -105.6453052450382017, -283.2934342122385942, -305.6734946699169768 ) ) ;
#52158=CARTESIAN_POINT ( 'NONE',  ( 37.34402547939911443, -279.4570430021292395, -262.9665257646339001 ) ) ;
#52160=CARTESIAN_POINT ( 'NONE',  ( 2.468690539327602629, -291.3933823303848385, -208.6384096722917718 ) ) ;
#52161=CARTESIAN_POINT ( 'NONE',  ( -111.2212738335056486, -282.7924386095645559, -262.5977180442585563 ) ) ;
#52164=CARTESIAN_POINT ( 'NONE',  ( 16.32392896252184045, -290.8135480300771860, -217.8939504077496281 ) ) ;
#52165=CARTESIAN_POINT ( 'NONE',  ( -107.0127715417791592, -279.8302058885995507, -294.8548815900806517 ) ) ;
#52166=CARTESIAN_POINT ( 'NONE',  ( -10.82500723068411652, -283.9191455476691885, -342.2845326428032990 ) ) ;
#52167=CARTESIAN_POINT ( 'NONE',  ( 17.06994838128405334, -272.8998257158513638, -217.8580643132578416 ) ) ;
#52168=CARTESIAN_POINT ( 'NONE',  ( -62.56287270591849392, -285.7147473351174085, -201.8025206523164456 ) ) ;
#52170=CARTESIAN_POINT ( 'NONE',  ( 33.46976579056012469, -277.2406190765233873, -290.4350344631953362 ) ) ;
#52171=CARTESIAN_POINT ( 'NONE',  ( -36.45397935899352149, -277.8436159201864371, -343.5297038731206385 ) ) ;
#52173=CARTESIAN_POINT ( 'NONE',  ( -92.46748606184532093, -287.2637938610868105, -219.4307883144246318 ) ) ;
#52176=CARTESIAN_POINT ( 'NONE',  ( -114.3096149042389129, -296.4308450680517808, -266.7331628054485577 ) ) ;
#52177=CARTESIAN_POINT ( 'NONE',  ( -27.64735173274831936, -288.1557945735045223, -196.3485081770893430 ) ) ;
#52179=CARTESIAN_POINT ( 'NONE',  ( -2.602324593224659921, -289.9809262143061233, -198.2974183793908196 ) ) ;
#52180=CARTESIAN_POINT ( 'NONE',  ( -103.1392927002287365, -277.9894602966368780, -230.8603112855608401 ) ) ;
#52181=CARTESIAN_POINT ( 'NONE',  ( -58.69477911175830087, -290.1803518300372957, -197.2140986884464837 ) ) ;
#52182=CARTESIAN_POINT ( 'NONE',  ( -62.82058670764900654, -287.2346241981953199, -201.1580543353766188 ) ) ;
#52184=CARTESIAN_POINT ( 'NONE',  ( -60.06577537862530392, -281.5138556556065055, -199.8685097336237391 ) ) ;
#52185=CARTESIAN_POINT ( 'NONE',  ( 38.09624322570690680, -289.1346567075709117, -282.8374009581613109 ) ) ;
#52186=CARTESIAN_POINT ( 'NONE',  ( -29.20297966300415382, -284.9493176891267581, -344.9701106552531087 ) ) ;
#52187=CARTESIAN_POINT ( 'NONE',  ( 20.82164410018379641, -276.4008681280163842, -320.8392292823531307 ) ) ;
#52188=CARTESIAN_POINT ( 'NONE',  ( -44.70683831060090796, -295.9787234687999558, -196.0290414908731975 ) ) ;
#52189=CARTESIAN_POINT ( 'NONE',  ( -68.67058123078733445, -279.4849870662441731, -200.0082564251513304 ) ) ;
#52190=CARTESIAN_POINT ( 'NONE',  ( -106.1015046846996768, -298.8473535845913034, -241.8408887985676472 ) ) ;
#52192=CARTESIAN_POINT ( 'NONE',  ( -54.49178911615187815, -276.3376638359844151, -195.3683826091709363 ) ) ;
#52193=CARTESIAN_POINT ( 'NONE',  ( -2.995253580873811217, -272.7394940055267512, -202.5653733163308061 ) ) ;
#52195=CARTESIAN_POINT ( 'NONE',  ( -69.76195965430177637, -279.1209892610443717, -204.8727229373165812 ) ) ;
#52196=CARTESIAN_POINT ( 'NONE',  ( -83.35390454241726843, -274.6426911799892423, -209.0502436942386169 ) ) ;
#52197=CARTESIAN_POINT ( 'NONE',  ( 35.10960980415642751, -280.2881446735348732, -244.8324595290386583 ) ) ;
#52198=CARTESIAN_POINT ( 'NONE',  ( -58.96405129887069307, -291.0957696810806965, -341.1991667748499140 ) ) ;
#52199=CARTESIAN_POINT ( 'NONE',  ( -113.5424571414612842, -274.1878846411663062, -267.5437725780381584 ) ) ;
#52200=CARTESIAN_POINT ( 'NONE',  ( -91.36641757709223555, -298.5090483409860553, -216.0533043404143712 ) ) ;
#52201=CARTESIAN_POINT ( 'NONE',  ( -36.20316001007722662, -294.0665827789429727, -195.5236517174657536 ) ) ;
#52202=CARTESIAN_POINT ( 'NONE',  ( 28.45519661566180858, -280.0264956285664084, -306.0093550024717501 ) ) ;
#52203=CARTESIAN_POINT ( 'NONE',  ( 19.92860285743860516, -282.8106810769454000, -222.7868839446012714 ) ) ;
#52204=CARTESIAN_POINT ( 'NONE',  ( -95.88742105534811344, -271.2113545362793730, -224.0551208737960849 ) ) ;
#52205=CARTESIAN_POINT ( 'NONE',  ( -85.58003301266370499, -285.3069691600299507, -329.3484357205357469 ) ) ;
#52206=CARTESIAN_POINT ( 'NONE',  ( -42.70017646613053586, -288.0415252847731722, -343.5249502488745179 ) ) ;
#52207=CARTESIAN_POINT ( 'NONE',  ( 104.5201122122490460, 115.5852336579065565, -282.7634610850568038 ) ) ;
#52209=CARTESIAN_POINT ( 'NONE',  ( -57.15574300866157387, -287.8775095005001390, -344.2128920102268239 ) ) ;
#52210=CARTESIAN_POINT ( 'NONE',  ( -23.78541194014374227, -288.5409996045896150, -342.1645875696741541 ) ) ;
#52212=CARTESIAN_POINT ( 'NONE',  ( -7.476245505745178654, -287.5141898714292097, -199.6679687439149689 ) ) ;
#52213=CARTESIAN_POINT ( 'NONE',  ( 17.29855352770658783, -275.1927481479630728, -221.8452031013103749 ) ) ;
#52214=CARTESIAN_POINT ( 'NONE',  ( 39.29747719142622486, -292.5078404395451912, -273.1769675353560274 ) ) ;
#52215=CARTESIAN_POINT ( 'NONE',  ( 2.049056795971745615, -283.1906971140581959, -336.4041422583042049 ) ) ;
#52216=CARTESIAN_POINT ( 'NONE',  ( 37.19251928460440837, -283.2793807728432967, -286.7726113737907099 ) ) ;
#52217=CARTESIAN_POINT ( 'NONE',  ( -63.90073798441968478, -283.7225086566691061, -342.6131892306777331 ) ) ;
#52218=CARTESIAN_POINT ( 'NONE',  ( 30.03937217322215503, -281.5080590244675705, -242.2207807027742206 ) ) ;
#52219=CARTESIAN_POINT ( 'NONE',  ( -102.0455923789670294, -293.6237833571632905, -301.4846348637937581 ) ) ;
#52220=CARTESIAN_POINT ( 'NONE',  ( -99.79643602748313924, -248.2790206999385418, -334.3247771912284065 ) ) ;
#52222=CARTESIAN_POINT ( 'NONE',  ( -105.9420827738617419, -280.1586023711414555, -300.3909596906286197 ) ) ;
#52223=CARTESIAN_POINT ( 'NONE',  ( -113.0788633804183974, -270.3086391544106846, -296.1849204825808783 ) ) ;
#52224=CARTESIAN_POINT ( 'NONE',  ( -35.80457197443260497, -297.4204801403503211, -197.2593596909151188 ) ) ;
#52225=CARTESIAN_POINT ( 'NONE',  ( 37.72250070525240062, -293.2718129439862196, -287.2993256315229473 ) ) ;
#52226=CARTESIAN_POINT ( 'NONE',  ( -38.36988802025361167, -140.4513536128933708, -361.1260187711026219 ) ) ;
#52227=CARTESIAN_POINT ( 'NONE',  ( -36.17716605900034921, -296.6411970502992403, -193.9506182268528107 ) ) ;
#52228=CARTESIAN_POINT ( 'NONE',  ( -48.19858638698259767, -287.5923142738738534, -343.4097444477936278 ) ) ;
#52229=CARTESIAN_POINT ( 'NONE',  ( -95.73053935388782065, -297.7768386694273204, -316.2044265199338611 ) ) ;
#52230=CARTESIAN_POINT ( 'NONE',  ( 16.32319716211788929, -288.1495819208435023, -220.1297815052000999 ) ) ;
#52232=CARTESIAN_POINT ( 'NONE',  ( -71.95717423407748470, -296.4398537462719219, -338.8781900615294376 ) ) ;
#52233=CARTESIAN_POINT ( 'NONE',  ( -109.4828918771271447, -285.1979156292162543, -258.7216874095224739 ) ) ;
#52234=CARTESIAN_POINT ( 'NONE',  ( -107.4036183759300229, -295.7457955590860479, -239.2568745477867367 ) ) ;
#52235=CARTESIAN_POINT ( 'NONE',  ( 29.33044666762119235, -293.8576570820348479, -232.1644733426883533 ) ) ;
#52237=CARTESIAN_POINT ( 'NONE',  ( 28.05692516249162693, -294.5760738690443077, -310.9895673690463127 ) ) ;
#52238=CARTESIAN_POINT ( 'NONE',  ( -91.67457854090307023, -291.4167528935680593, -221.5885660294431716 ) ) ;
#52241=CARTESIAN_POINT ( 'NONE',  ( -32.04153465397340028, -299.9782412895974630, -194.5946519202969966 ) ) ;
#52242=CARTESIAN_POINT ( 'NONE',  ( 36.10834357068222999, -274.6219025954721928, -292.1582231066766440 ) ) ;
#52245=CARTESIAN_POINT ( 'NONE',  ( 21.67938326231145396, -275.7245556980903416, -319.7173599271187641 ) ) ;
#52246=CARTESIAN_POINT ( 'NONE',  ( -59.69880733101615533, -272.1576865900379971, -199.9755513670415041 ) ) ;
#52247=CARTESIAN_POINT ( 'NONE',  ( -93.15247091760456044, -281.0997360828169462, -221.3925815079106769 ) ) ;
#52248=CARTESIAN_POINT ( 'NONE',  ( 29.12608476439344329, -274.1339236686507093, -303.5359506368039320 ) ) ;
#52249=CARTESIAN_POINT ( 'NONE',  ( -106.6029141340631128, -273.9499625306101507, -246.3379977065959281 ) ) ;
#52250=CARTESIAN_POINT ( 'NONE',  ( -83.34766954163977459, -274.3447446375503205, -213.3798997989499071 ) ) ;
#52251=CARTESIAN_POINT ( 'NONE',  ( -112.0758621855516566, -274.4899798628269991, -256.3400642169655157 ) ) ;
#52252=CARTESIAN_POINT ( 'NONE',  ( -36.92299820561722612, -272.0775152233853760, -194.9943032149767248 ) ) ;
#52253=CARTESIAN_POINT ( 'NONE',  ( -28.87594990684027252, -295.5935514561290347, -343.0222835012285145 ) ) ;
#52254=CARTESIAN_POINT ( 'NONE',  ( -39.72616871266622240, -293.6573735594915320, -343.9242381158488797 ) ) ;
#52256=CARTESIAN_POINT ( 'NONE',  ( 27.60025669824054972, -276.5867490848583543, -311.7163031328891520 ) ) ;
#52257=CARTESIAN_POINT ( 'NONE',  ( -19.27367601625923754, -274.4577180917642636, -199.5800088567652608 ) ) ;
#52259=CARTESIAN_POINT ( 'NONE',  ( -78.24457982879074791, -284.1990046914297636, -205.7062441964519337 ) ) ;
#52260=CARTESIAN_POINT ( 'NONE',  ( -111.0949054073396383, -298.7390324594260278, -255.7864317656489277 ) ) ;
#52262=CARTESIAN_POINT ( 'NONE',  ( -62.60906559795499504, -284.9120442018341350, -201.6473387331715514 ) ) ;
#52263=CARTESIAN_POINT ( 'NONE',  ( -78.18542002612213082, -281.5999099524242979, -333.4627738237135759 ) ) ;
#52264=CARTESIAN_POINT ( 'NONE',  ( -107.2283657833909842, -276.4704778003267052, -294.8852725946598525 ) ) ;
#52265=CARTESIAN_POINT ( 'NONE',  ( -74.32497404582281320, -276.1290275065254605, -333.9819665128457018 ) ) ;
#52266=CARTESIAN_POINT ( 'NONE',  ( -79.22866505866824127, -281.4875137572931294, -208.0864290716669416 ) ) ;
#52267=CARTESIAN_POINT ( 'NONE',  ( 29.44099802228070573, -276.3474348901758049, -239.7882390472778980 ) ) ;
#52269=CARTESIAN_POINT ( 'NONE',  ( -97.17213311375004992, -271.5898310211052831, -223.1725631474939178 ) ) ;
#52271=CARTESIAN_POINT ( 'NONE',  ( -71.69226807176488592, -281.5995509806118093, -203.4882545163977170 ) ) ;
#52273=CARTESIAN_POINT ( 'NONE',  ( -62.74083993830809192, -287.6442476405991329, -199.1979400461866305 ) ) ;
#52275=CARTESIAN_POINT ( 'NONE',  ( -107.9953965008220251, -288.2242014640054322, -295.6740867377243376 ) ) ;
#52277=CARTESIAN_POINT ( 'NONE',  ( -86.35410667279552399, -296.1483796986403263, -215.7267468545307167 ) ) ;
#52278=CARTESIAN_POINT ( 'NONE',  ( -111.1994714745900978, -288.7887144184945782, -262.8848160411922095 ) ) ;
#52279=CARTESIAN_POINT ( 'NONE',  ( 176.3450237082407170, 252.7779579681928510, -162.7338909149122799 ) ) ;
#52280=CARTESIAN_POINT ( 'NONE',  ( -36.42824076990669369, -296.0634301785021307, -195.3614206927910288 ) ) ;
#52281=CARTESIAN_POINT ( 'NONE',  ( 33.39228819982854901, -286.4003668629079584, -299.1271209836299363 ) ) ;
#52282=CARTESIAN_POINT ( 'NONE',  ( -65.48099292909800795, -283.9291461649952453, -199.7627751490661581 ) ) ;
#52283=CARTESIAN_POINT ( 'NONE',  ( -64.07161016993896396, -291.6935386965579937, -202.4173861224734310 ) ) ;
#52284=CARTESIAN_POINT ( 'NONE',  ( 33.53178848499534581, -283.2371216244124525, -290.1682765343626897 ) ) ;
#52285=CARTESIAN_POINT ( 'NONE',  ( 35.86453168550522719, -282.3674224830651838, -271.3056627519301287 ) ) ;
#52286=CARTESIAN_POINT ( 'NONE',  ( -36.08835932941323676, -291.0164317800134768, -345.7187284094392794 ) ) ;
#52287=CARTESIAN_POINT ( 'NONE',  ( -105.5921610927945693, -273.3461394712598462, -234.6422622789075945 ) ) ;
#52289=CARTESIAN_POINT ( 'NONE',  ( -74.96822895289646738, -287.6290991539262905, -335.8863690472172152 ) ) ;
#52290=CARTESIAN_POINT ( 'NONE',  ( 26.93056093854354671, -274.9945429980666063, -227.9573863380029195 ) ) ;
#52291=CARTESIAN_POINT ( 'NONE',  ( -70.98410693037212127, -293.5858316258687069, -203.7275283237966335 ) ) ;
#52293=CARTESIAN_POINT ( 'NONE',  ( -37.37352853689063892, -276.5519495502701943, -195.3611179825600175 ) ) ;
#52295=CARTESIAN_POINT ( 'NONE',  ( -74.45373774874848039, -275.5444467006205969, -335.7272031572723563 ) ) ;
#52298=CARTESIAN_POINT ( 'NONE',  ( -36.53050614715974831, -296.4620263312577890, -194.1613290880058287 ) ) ;
#52299=CARTESIAN_POINT ( 'NONE',  ( 19.08281540511503138, -274.2429869052108984, -223.8835242907718452 ) ) ;
#52300=CARTESIAN_POINT ( 'NONE',  ( -109.3924920092680537, -292.2744608631003302, -254.8888478261050352 ) ) ;
#52301=CARTESIAN_POINT ( 'NONE',  ( -37.56265529339778908, -292.9906090994365968, -197.1136725838293273 ) ) ;
#52302=CARTESIAN_POINT ( 'NONE',  ( -110.8769012073965854, -286.1972786594106992, -279.2013363439521072 ) ) ;
#52303=CARTESIAN_POINT ( 'NONE',  ( 35.81091884827876015, -295.2586736805342298, -292.6153884610375258 ) ) ;
#52304=CARTESIAN_POINT ( 'NONE',  ( 38.33125616875052089, -295.0091159676366601, -281.6261949062842973 ) ) ;
#52305=CARTESIAN_POINT ( 'NONE',  ( 35.62139719961320594, -293.3548549169972262, -268.0402490001837918 ) ) ;
#52306=CARTESIAN_POINT ( 'NONE',  ( 35.65105399330508362, -289.3302962857743523, -253.0703076809304264 ) ) ;
#52307=CARTESIAN_POINT ( 'NONE',  ( 23.40422678958352876, -282.3511815743451052, -317.6997836591381201 ) ) ;
#52308=CARTESIAN_POINT ( 'NONE',  ( -75.03984912860983059, -295.6343364933470639, -204.8170072491263056 ) ) ;
#52309=CARTESIAN_POINT ( 'NONE',  ( -83.27417751675818636, -285.2759011029294243, -208.4948925254547873 ) ) ;
#52310=CARTESIAN_POINT ( 'NONE',  ( 36.64761386858147318, -277.4047072812848000, -260.4905447091874748 ) ) ;
#52311=CARTESIAN_POINT ( 'NONE',  ( -70.14620202639585500, -284.4049355590382220, -204.6889301401840555 ) ) ;
#52312=CARTESIAN_POINT ( 'NONE',  ( 35.44225815491537901, -285.3195529179867549, -252.2642655184450575 ) ) ;
#52313=CARTESIAN_POINT ( 'NONE',  ( -112.0150127718244022, -276.8546106223477068, -257.5469906024507623 ) ) ;
#52314=CARTESIAN_POINT ( 'NONE',  ( -96.12512592106646991, -239.9971452530988358, -342.0757611934672582 ) ) ;
#52315=CARTESIAN_POINT ( 'NONE',  ( -110.2892526500924504, -284.1244694689802941, -265.4548301130283789 ) ) ;
#52316=CARTESIAN_POINT ( 'NONE',  ( 39.24300616143346332, -282.7157161040599931, -267.0591067904675810 ) ) ;
#52317=CARTESIAN_POINT ( 'NONE',  ( -65.37231033901473154, -288.4683628268691677, -341.8813056416111635 ) ) ;
#52318=CARTESIAN_POINT ( 'NONE',  ( -59.41361302702041769, -278.9334098876110488, -343.2944510668927478 ) ) ;
#52319=CARTESIAN_POINT ( 'NONE',  ( -14.71942797581068163, -278.0802905493025605, -343.5023688635482131 ) ) ;
#52320=CARTESIAN_POINT ( 'NONE',  ( -108.8868216375025071, -278.5775993403344160, -255.7967833659311907 ) ) ;
#52321=CARTESIAN_POINT ( 'NONE',  ( -108.7778476816431521, -274.8144592959327497, -248.5338331468987860 ) ) ;
#52322=CARTESIAN_POINT ( 'NONE',  ( 34.43548766501601932, -285.2782388294936595, -249.1483444866740058 ) ) ;
#52324=CARTESIAN_POINT ( 'NONE',  ( -71.52909317333094918, -291.0963266965711114, -338.4615039932623404 ) ) ;
#52325=CARTESIAN_POINT ( 'NONE',  ( 19.06215812625640282, -293.1338711974787543, -317.1887898077374075 ) ) ;
#52327=CARTESIAN_POINT ( 'NONE',  ( 35.44517167726820617, -293.2959459824859891, -276.2056692489124430 ) ) ;
#52328=CARTESIAN_POINT ( 'NONE',  ( -97.23083220015577410, -292.2760525810689956, -222.4572103016551239 ) ) ;
#52329=CARTESIAN_POINT ( 'NONE',  ( -93.17341507491963171, -279.8734165986069797, -223.1538078118960868 ) ) ;
#52330=CARTESIAN_POINT ( 'NONE',  ( -37.24013962337803463, -296.9737320793004756, -193.6694850293974923 ) ) ;
#52331=CARTESIAN_POINT ( 'NONE',  ( 30.27701715302099572, -288.6791610273500055, -307.0924682078160686 ) ) ;
#52332=CARTESIAN_POINT ( 'NONE',  ( -28.97525765558017596, -289.2822734023411044, -346.9374817757678215 ) ) ;
#52333=CARTESIAN_POINT ( 'NONE',  ( -87.71215491142604037, -285.6579220070659062, -217.4942590666043429 ) ) ;
#52335=CARTESIAN_POINT ( 'NONE',  ( 101.3871863598238150, 116.2727258721154016, -280.9442760304585818 ) ) ;
#52336=CARTESIAN_POINT ( 'NONE',  ( 64.67481406031001256, 46.43102927970478078, -315.2674948880320471 ) ) ;
#52337=CARTESIAN_POINT ( 'NONE',  ( 0.9472411158466204073, -275.7245445414006895, -332.7629115109273243 ) ) ;
#52338=CARTESIAN_POINT ( 'NONE',  ( -109.7996693342661558, -277.3261591556681651, -281.4997342510224598 ) ) ;
#52339=CARTESIAN_POINT ( 'NONE',  ( 99.05675807372718111, -299.2246248443447598, -193.4335806325171063 ) ) ;
#52340=CARTESIAN_POINT ( 'NONE',  ( 198.1527406508571403, 281.8181044100605277, -110.6140813440772206 ) ) ;
#52341=CARTESIAN_POINT ( 'NONE',  ( -34.32739795775894720, -275.6998269976061238, -346.8085656587232961 ) ) ;
#52343=CARTESIAN_POINT ( 'NONE',  ( 34.53530344557626819, -295.6289451990185171, -295.1734719724599358 ) ) ;
#52344=CARTESIAN_POINT ( 'NONE',  ( -6.020930759994383763, -292.9676237087123241, -204.3397661662521614 ) ) ;
#52345=CARTESIAN_POINT ( 'NONE',  ( -60.11001654370966918, -298.5673208123796485, -196.9179546232559801 ) ) ;
#52346=CARTESIAN_POINT ( 'NONE',  ( 24.64536334402888684, -286.7792410129834479, -309.8433600644539752 ) ) ;
#52347=CARTESIAN_POINT ( 'NONE',  ( -110.0082557544233026, -273.5211440984238607, -245.2039225932294642 ) ) ;
#52348=CARTESIAN_POINT ( 'NONE',  ( -101.4663034235060763, -296.2426583400958862, -305.2471503836522970 ) ) ;
#52349=VERTEX_POINT ( 'NONE', #88515 ) ;
#52351=CARTESIAN_POINT ( 'NONE',  ( -111.8746498547990882, -280.3140671629762437, -282.7769789732384993 ) ) ;
#52352=CARTESIAN_POINT ( 'NONE',  ( -52.91129460743638191, -282.7540768230894059, -345.7621972615469303 ) ) ;
#52353=CARTESIAN_POINT ( 'NONE',  ( -102.1236871655778486, -279.1663604890888450, -304.6761325999314636 ) ) ;
#52354=CARTESIAN_POINT ( 'NONE',  ( -72.35357213905712115, -279.2690556255807337, -337.8155466222253267 ) ) ;
#52355=CARTESIAN_POINT ( 'NONE',  ( -19.08127780748096214, -272.7711875065089089, -198.9130584666494315 ) ) ;
#52358=CARTESIAN_POINT ( 'NONE',  ( -37.01045736687348153, -280.2230949378517835, -197.3618694742876301 ) ) ;
#52359=CARTESIAN_POINT ( 'NONE',  ( -4.055529868744314648, -277.4271652916872313, -339.6301157917125124 ) ) ;
#52361=CARTESIAN_POINT ( 'NONE',  ( -2.376937179892249397, -278.5896319205613167, -336.7121993858632436 ) ) ;
#52362=CARTESIAN_POINT ( 'NONE',  ( -31.51346126257525881, -275.5547949551692000, -346.6015131596551555 ) ) ;
#52365=CARTESIAN_POINT ( 'NONE',  ( 22.12090015254715070, -284.1641002632627533, -316.6702701252370957 ) ) ;
#52366=CARTESIAN_POINT ( 'NONE',  ( -72.69603300476974539, -290.7687560346113287, -206.2520816521913218 ) ) ;
#52367=CARTESIAN_POINT ( 'NONE',  ( -23.79569790784137240, -285.5693231229910225, -194.6114066283914497 ) ) ;
#52368=CARTESIAN_POINT ( 'NONE',  ( -70.69132299255099383, -281.7379893869597822, -336.4493165470716463 ) ) ;
#52369=CARTESIAN_POINT ( 'NONE',  ( -13.35431244945859142, -281.3092974053558919, -339.9851159264639477 ) ) ;
#52370=CARTESIAN_POINT ( 'NONE',  ( -1.471439006538290517, -284.6110733983196042, -205.0756838971511797 ) ) ;
#52371=CARTESIAN_POINT ( 'NONE',  ( -5.399483264460136489, -281.6871709029481394, -204.2791591125973696 ) ) ;
#52372=CARTESIAN_POINT ( 'NONE',  ( -109.8772534207676301, -270.7993796934649140, -251.0944607303940472 ) ) ;
#52373=CARTESIAN_POINT ( 'NONE',  ( 20.98438742906629528, -280.6192550429955190, -319.3969000997288958 ) ) ;
#52374=CARTESIAN_POINT ( 'NONE',  ( 26.34034625178250622, -295.0190670008250322, -230.6448913260919653 ) ) ;
#52375=CARTESIAN_POINT ( 'NONE',  ( -91.03709241739313995, -278.4914154407168780, -320.0401568655017854 ) ) ;
#52376=CARTESIAN_POINT ( 'NONE',  ( -67.78222292530867321, -287.6537837865798792, -201.6200634679121606 ) ) ;
#52378=CARTESIAN_POINT ( 'NONE',  ( -98.06227083150329804, -293.0817304693117649, -225.3691499501454416 ) ) ;
#52379=CARTESIAN_POINT ( 'NONE',  ( 17.03074158712967190, -274.2768656515434600, -322.0199819911745180 ) ) ;
#52380=CARTESIAN_POINT ( 'NONE',  ( -6.993132136467158588, -287.8611281778326543, -340.9665677939642592 ) ) ;
#52381=CARTESIAN_POINT ( 'NONE',  ( 30.60013466689604655, -291.5677956961148993, -241.4145391574006112 ) ) ;
#52382=CARTESIAN_POINT ( 'NONE',  ( 104.1964229570258311, -299.5541904835127980, -195.3611179825600175 ) ) ;
#52383=CARTESIAN_POINT ( 'NONE',  ( -110.4549175772959870, -277.3411416829256382, -262.4111418263187829 ) ) ;
#52384=CARTESIAN_POINT ( 'NONE',  ( -109.9829726674479957, -294.8909945743895378, -254.9994061884682708 ) ) ;
#52385=CARTESIAN_POINT ( 'NONE',  ( -110.1088799110917620, -291.7311299096236326, -280.7556769328962787 ) ) ;
#52387=CARTESIAN_POINT ( 'NONE',  ( 144.7857639756989272, -299.5541904835127980, -193.4639945212225882 ) ) ;
#52388=CARTESIAN_POINT ( 'NONE',  ( 6.117384586893342302, -291.1101648205416836, -207.6393856486895686 ) ) ;
#52389=CARTESIAN_POINT ( 'NONE',  ( 32.15957837496912930, -289.4791597784695227, -295.1807211375624433 ) ) ;
#52390=CARTESIAN_POINT ( 'NONE',  ( -90.90040963242593364, -288.0390466126032720, -324.3372796021014324 ) ) ;
#52391=CARTESIAN_POINT ( 'NONE',  ( 5.050100288672720872, -288.0627099524260188, -210.1463796360941387 ) ) ;
#52393=CARTESIAN_POINT ( 'NONE',  ( 9.125190330691086871, -287.5122677333324077, -213.8506780841118768 ) ) ;
#52394=CARTESIAN_POINT ( 'NONE',  ( -5.181125409545572325, -296.6108969255783450, -338.5229464285263248 ) ) ;
#52396=CARTESIAN_POINT ( 'NONE',  ( -65.28778883781605202, -290.6143442295254999, -341.7405471317194952 ) ) ;
#52397=CARTESIAN_POINT ( 'NONE',  ( -101.9873113512920071, -277.0893845098545398, -231.5382513952465615 ) ) ;
#52398=CARTESIAN_POINT ( 'NONE',  ( -71.55763747030638910, -277.8250961219876558, -339.3177269728706165 ) ) ;
#52399=CARTESIAN_POINT ( 'NONE',  ( -50.93172707210779038, -279.5497596932047486, -194.5913650523636989 ) ) ;
#52400=CARTESIAN_POINT ( 'NONE',  ( -61.06194253584868648, -299.7227565946490131, -199.5307572127530591 ) ) ;
#52401=CARTESIAN_POINT ( 'NONE',  ( -111.1570253307531146, -282.7234030645911957, -257.0112620146076097 ) ) ;
#52402=CARTESIAN_POINT ( 'NONE',  ( -110.3557390660489546, -272.8426144905440651, -270.3648162637165910 ) ) ;
#52403=CARTESIAN_POINT ( 'NONE',  ( -43.83593020672741147, -278.1089255674569927, -196.3594393412735712 ) ) ;
#52405=CARTESIAN_POINT ( 'NONE',  ( -108.7882805279044049, -282.2570618759681906, -293.2155039428967598 ) ) ;
#52407=CARTESIAN_POINT ( 'NONE',  ( 32.37836650704268493, -274.4314699551513854, -301.3743419256232983 ) ) ;
#52409=CARTESIAN_POINT ( 'NONE',  ( -100.5009135111393448, -298.5909439488834209, -232.2931477166583250 ) ) ;
#52410=CARTESIAN_POINT ( 'NONE',  ( -79.00338075339101351, -282.5202507145826871, -334.7489807884668949 ) ) ;
#52411=CARTESIAN_POINT ( 'NONE',  ( -109.1129221040446993, -297.3009943647230671, -284.9940441137471794 ) ) ;
#52412=CARTESIAN_POINT ( 'NONE',  ( -78.53925624087929691, -274.9343058753559035, -206.0076591605692613 ) ) ;
#52413=CARTESIAN_POINT ( 'NONE',  ( -87.34469137041550368, -272.9985724966560952, -217.0773419629727528 ) ) ;
#52414=CARTESIAN_POINT ( 'NONE',  ( 31.68679697324006739, -295.1675051200704729, -240.9014555438631362 ) ) ;
#52415=CARTESIAN_POINT ( 'NONE',  ( 18.64627367818471271, -288.4407241664070511, -323.2226994342595958 ) ) ;
#52416=CARTESIAN_POINT ( 'NONE',  ( -90.03608180449151632, -277.3949769852837335, -216.1345633064935612 ) ) ;
#52417=CARTESIAN_POINT ( 'NONE',  ( -99.87150825291023182, -289.7896485194476099, -315.3172497210196639 ) ) ;
#52418=CARTESIAN_POINT ( 'NONE',  ( -13.22165112776366236, -287.7897306041386400, -339.5104613209703643 ) ) ;
#52419=CARTESIAN_POINT ( 'NONE',  ( -17.14018917502054862, -290.3127891147919968, -198.1330098721718400 ) ) ;
#52422=CARTESIAN_POINT ( 'NONE',  ( -106.6276633170962640, -290.3674417480760894, -247.1782849673035116 ) ) ;
#52424=CARTESIAN_POINT ( 'NONE',  ( -68.41652929817374229, -286.5950465038032462, -200.1529442076306111 ) ) ;
#52425=CARTESIAN_POINT ( 'NONE',  ( -67.68488546085839630, -285.9805209788416391, -333.4427485647536855 ) ) ;
#52426=CARTESIAN_POINT ( 'NONE',  ( -64.19513912797437172, -294.4528645062738406, -342.2757411595842427 ) ) ;
#52427=CARTESIAN_POINT ( 'NONE',  ( -35.89163966851172916, -284.3495241195543031, -346.8672589026031687 ) ) ;
#52428=CARTESIAN_POINT ( 'NONE',  ( -97.35473082005590584, -284.9647930023663776, -228.7765863489638321 ) ) ;
#52429=CARTESIAN_POINT ( 'NONE',  ( 32.99318850367090050, -277.1481589334998716, -291.7178459323778839 ) ) ;
#52430=CARTESIAN_POINT ( 'NONE',  ( -32.01530749876538096, -290.1397599142433705, -195.8936879466484129 ) ) ;
#52431=CARTESIAN_POINT ( 'NONE',  ( 24.13441779724263014, -273.7944709788256432, -230.2635191818106648 ) ) ;
#52432=ORIENTED_EDGE ( 'NONE', *, *, #7938, .T. ) ;
#52433=CARTESIAN_POINT ( 'NONE',  ( 193.6056169066500274, 279.7126221763799094, -126.0203154767880989 ) ) ;
#52434=CARTESIAN_POINT ( 'NONE',  ( -82.36865183200259821, -287.3521690720007769, -211.0830628928584929 ) ) ;
#52435=CARTESIAN_POINT ( 'NONE',  ( -113.2975372549769730, -297.7660238535736426, -259.6733947777154299 ) ) ;
#52436=CARTESIAN_POINT ( 'NONE',  ( -39.98590122183763640, -286.6694679753457535, -197.3070224846128440 ) ) ;
#52437=CARTESIAN_POINT ( 'NONE',  ( -91.17261100891231251, -276.8530948807335221, -325.1626483146377495 ) ) ;
#52438=CARTESIAN_POINT ( 'NONE',  ( 23.88902485567300360, -293.5825681142474082, -223.8194447735538688 ) ) ;
#52439=CARTESIAN_POINT ( 'NONE',  ( -1.532106799640005512, -284.6613288703608760, -203.5930229971604319 ) ) ;
#52440=CARTESIAN_POINT ( 'NONE',  ( 11.18827304455897576, -294.7345294640700786, -330.1841937565848752 ) ) ;
#52441=CARTESIAN_POINT ( 'NONE',  ( -28.10788012022588589, -292.5057275594162434, -197.8753908599403530 ) ) ;
#52444=CARTESIAN_POINT ( 'NONE',  ( 103.5299684544230132, 114.3122098872502903, -279.6362027374893273 ) ) ;
#52445=CARTESIAN_POINT ( 'NONE',  ( -49.25574556654544267, -287.4232086373899051, -194.9370262290599953 ) ) ;
#52446=CARTESIAN_POINT ( 'NONE',  ( -72.08107566293803359, -274.9809262143061233, -342.4248175857292154 ) ) ;
#52448=CARTESIAN_POINT ( 'NONE',  ( -59.05273952577334740, -282.2599783257348349, -340.4348910940807968 ) ) ;
#52449=CARTESIAN_POINT ( 'NONE',  ( -106.1547724962572943, -278.6641666460085389, -235.7387116239097509 ) ) ;
#52450=CARTESIAN_POINT ( 'NONE',  ( 3.688413325188839575, -282.6053565908349015, -207.7165416612079127 ) ) ;
#52451=CARTESIAN_POINT ( 'NONE',  ( 201.3362163961940894, 286.9516950286333667, -97.02954773690071022 ) ) ;
#52452=CARTESIAN_POINT ( 'NONE',  ( -76.47187148977623394, -282.1391075178447068, -336.0535317128639576 ) ) ;
#52453=CARTESIAN_POINT ( 'NONE',  ( 27.81515970384150904, -285.0838445413864406, -233.8351088032227381 ) ) ;
#52454=CARTESIAN_POINT ( 'NONE',  ( -4.385165432208308012, -276.3422400265334318, -202.1253504088959687 ) ) ;
#52455=CARTESIAN_POINT ( 'NONE',  ( -99.95276298598618325, -297.5633347333634902, -232.6084591510642383 ) ) ;
#52456=CARTESIAN_POINT ( 'NONE',  ( 26.21077360547631230, -292.7399702983381644, -307.2708261826982152 ) ) ;
#52457=CARTESIAN_POINT ( 'NONE',  ( -99.35059563998457577, -279.8085729565765973, -224.8613183859665128 ) ) ;
#52458=CARTESIAN_POINT ( 'NONE',  ( -29.71342446088390332, -276.9530217965064480, -343.0123641852457581 ) ) ;
#52459=CARTESIAN_POINT ( 'NONE',  ( -114.0325882487032771, -273.6316498053999453, -270.3748343644707006 ) ) ;
#52460=CARTESIAN_POINT ( 'NONE',  ( -9.337548418294215224, -275.6148612043954245, -341.7562158312675820 ) ) ;
#52462=CARTESIAN_POINT ( 'NONE',  ( -81.72547948933774364, -275.6558952928574513, -330.8819030204403475 ) ) ;
#52463=CARTESIAN_POINT ( 'NONE',  ( -96.93638943534148211, -297.3314612213697501, -318.2052376438608121 ) ) ;
#52465=CARTESIAN_POINT ( 'NONE',  ( 85.37101130053461873, 80.99577858023421584, -298.5812782549759845 ) ) ;
#52466=CARTESIAN_POINT ( 'NONE',  ( -104.3904941616219020, -285.2345786884110908, -300.0037442383627990 ) ) ;
#52467=CARTESIAN_POINT ( 'NONE',  ( -55.43883764788490964, -285.0420571346780889, -344.1613051428636822 ) ) ;
#52468=CARTESIAN_POINT ( 'NONE',  ( -81.53361516298525657, -284.7810156614873449, -212.1291051941864225 ) ) ;
#52469=CARTESIAN_POINT ( 'NONE',  ( -96.74897785680791173, -276.3447727814161681, -314.1683300977257431 ) ) ;
#52470=CARTESIAN_POINT ( 'NONE',  ( -105.7447925619772207, -286.7947869522911333, -241.3865179874723026 ) ) ;
#52471=CARTESIAN_POINT ( 'NONE',  ( -41.06705688715102553, -278.4842915597006368, -196.7620047374585113 ) ) ;
#52472=CARTESIAN_POINT ( 'NONE',  ( 7.781432718798567016, -277.4992812736093697, -328.2023553674400205 ) ) ;
#52474=CARTESIAN_POINT ( 'NONE',  ( -59.50026941607413278, -274.2498251955237833, -200.6878495533262594 ) ) ;
#52475=CARTESIAN_POINT ( 'NONE',  ( 22.74263381614980162, -281.7121468791281700, -222.4441534035236998 ) ) ;
#52476=CARTESIAN_POINT ( 'NONE',  ( -24.53764419255239559, -283.3854183337106747, -346.2807504653053456 ) ) ;
#52480=CARTESIAN_POINT ( 'NONE',  ( 21.12168618264349007, -288.7544897939970951, -222.1704763067948249 ) ) ;
#52481=CARTESIAN_POINT ( 'NONE',  ( -107.9889243777503651, -296.0004932117155931, -251.2978366723341423 ) ) ;
#52482=CARTESIAN_POINT ( 'NONE',  ( -53.35997526107881583, -291.2006243366212743, -195.0954732389131152 ) ) ;
#52483=CARTESIAN_POINT ( 'NONE',  ( -10.48933625865610964, -287.1753552467637292, -339.0427926207207179 ) ) ;
#52484=CARTESIAN_POINT ( 'NONE',  ( -75.03316443154132287, -288.1395540132069755, -333.5797893537370555 ) ) ;
#52485=CARTESIAN_POINT ( 'NONE',  ( -81.73084617045694245, -286.6372058348181326, -211.9082804357130385 ) ) ;
#52486=CARTESIAN_POINT ( 'NONE',  ( -109.7922315684898962, -276.8018089381834557, -250.9229145987291076 ) ) ;
#52487=CARTESIAN_POINT ( 'NONE',  ( -37.52038352759148410, -287.4541964633958173, -346.5738469064804121 ) ) ;
#52488=CARTESIAN_POINT ( 'NONE',  ( 16.88731185407780444, -288.8241946479845979, -218.4768376535166681 ) ) ;
#52489=CARTESIAN_POINT ( 'NONE',  ( -104.8777640831846583, -288.1165675301670035, -303.4781241977089508 ) ) ;
#52490=CARTESIAN_POINT ( 'NONE',  ( -8.390229859892091469, -283.6048060190160527, -337.6308795245256533 ) ) ;
#52491=CARTESIAN_POINT ( 'NONE',  ( -106.6858705355471955, -292.9302466538327394, -241.3539730976788746 ) ) ;
#52492=CARTESIAN_POINT ( 'NONE',  ( 82.13248925020795355, -300.8400434547833129, -193.8278775912719993 ) ) ;
#52493=CARTESIAN_POINT ( 'NONE',  ( -36.93173961908839686, -299.9773941857664568, -194.8009771340476561 ) ) ;
#52494=CARTESIAN_POINT ( 'NONE',  ( 32.89246609102586660, -280.4788835943680283, -249.8729842779206933 ) ) ;
#52495=CARTESIAN_POINT ( 'NONE',  ( 10.57332435206023646, -278.7133933265144492, -212.5946024002020636 ) ) ;
#52496=CARTESIAN_POINT ( 'NONE',  ( 37.30069955418279193, -292.9785815627571424, -288.6554127986520939 ) ) ;
#52497=CARTESIAN_POINT ( 'NONE',  ( -101.5863744136171789, -271.2899124802105462, -233.5076557777846915 ) ) ;
#52498=CARTESIAN_POINT ( 'NONE',  ( -41.97007588457124427, -275.1907469621421569, -344.6699407535705859 ) ) ;
#52499=CARTESIAN_POINT ( 'NONE',  ( -34.26389064143585728, -296.3278239790259931, -343.7897947222320454 ) ) ;
#52501=CARTESIAN_POINT ( 'NONE',  ( -76.11793485492106015, -272.1197923858541685, -204.4591959942287644 ) ) ;
#52502=CARTESIAN_POINT ( 'NONE',  ( -96.63104715675237344, -294.1465636135915247, -317.9079980111311556 ) ) ;
#52503=CARTESIAN_POINT ( 'NONE',  ( -5.805447809746892673, -293.9003977623427772, -203.8578313996530085 ) ) ;
#52506=CARTESIAN_POINT ( 'NONE',  ( 34.64021106261860439, -294.1818450371639528, -257.2069297958757375 ) ) ;
#52507=FACE_OUTER_BOUND ( 'NONE', #41035, .T. ) ;
#52508=CARTESIAN_POINT ( 'NONE',  ( -108.4173242812693729, -282.8949612528888338, -245.3278910065147329 ) ) ;
#52509=CARTESIAN_POINT ( 'NONE',  ( -13.00824282778969199, -294.7271025551924026, -339.2393921967025676 ) ) ;
#52510=CARTESIAN_POINT ( 'NONE',  ( 35.60908434820196078, -281.8643890117031674, -295.1679019736784539 ) ) ;
#52511=CARTESIAN_POINT ( 'NONE',  ( 29.43749453929426352, -283.0057799938489325, -234.8963726358827273 ) ) ;
#52512=CARTESIAN_POINT ( 'NONE',  ( -78.50757173945926581, -285.1807392696085799, -205.3140941770536188 ) ) ;
#52513=CARTESIAN_POINT ( 'NONE',  ( -75.90301674169830903, -289.5362158941690609, -206.1675414716499404 ) ) ;
#52515=CARTESIAN_POINT ( 'NONE',  ( 18.15953800471899626, -285.5548350011254115, -222.1858541566391807 ) ) ;
#52516=CARTESIAN_POINT ( 'NONE',  ( -110.4911888724279549, -289.1798710766777276, -293.5704393380333954 ) ) ;
#52518=CARTESIAN_POINT ( 'NONE',  ( 4.284233765214266576, -296.0805612752665752, -331.3014333836509309 ) ) ;
#52519=CARTESIAN_POINT ( 'NONE',  ( -113.6426508860114808, -279.9258110459821296, -274.4563841396836779 ) ) ;
#52520=CARTESIAN_POINT ( 'NONE',  ( 7.898142624106161414, -292.4575675126488363, -330.6252319112911664 ) ) ;
#52521=CARTESIAN_POINT ( 'NONE',  ( 0.4145165703888758491, -280.2366115610857946, -207.8001399213111142 ) ) ;
#52522=CARTESIAN_POINT ( 'NONE',  ( -5.795760295993536815, -294.8153886807336903, -340.6025137875776636 ) ) ;
#52523=CARTESIAN_POINT ( 'NONE',  ( -110.4872666179995946, -282.3897395652596174, -289.3608382218905604 ) ) ;
#52525=CARTESIAN_POINT ( 'NONE',  ( -85.78348016252591890, -279.7225441534340575, -327.6863160859580262 ) ) ;
#52526=CARTESIAN_POINT ( 'NONE',  ( 3.939165828551679294, -293.5395901612440070, -330.8532542772171610 ) ) ;
#52527=CARTESIAN_POINT ( 'NONE',  ( -105.1774863663427766, -270.9772121210194769, -237.9831234665645638 ) ) ;
#52530=CARTESIAN_POINT ( 'NONE',  ( 22.63587310320395218, -282.9224551999581081, -225.9038460735818035 ) ) ;
#52531=CARTESIAN_POINT ( 'NONE',  ( -109.2037973509218176, -295.8851120624425448, -283.6148179868723673 ) ) ;
#52533=CARTESIAN_POINT ( 'NONE',  ( 31.95455697924147032, -273.4809262143061233, -303.7686719486574702 ) ) ;
#52534=CARTESIAN_POINT ( 'NONE',  ( -87.92237192801130163, -272.5633859286510869, -212.4478887049433808 ) ) ;
#52535=CARTESIAN_POINT ( 'NONE',  ( 25.45657604314171962, -289.4495432376438657, -314.1519322168629174 ) ) ;
#52536=CARTESIAN_POINT ( 'NONE',  ( -100.3050261004794947, -289.8770450642638252, -307.4014418045969705 ) ) ;
#52537=CARTESIAN_POINT ( 'NONE',  ( -57.31958891093502473, -281.3097404250933096, -199.4274044850136818 ) ) ;
#52538=CARTESIAN_POINT ( 'NONE',  ( -69.86164106181914235, -275.2166414825958896, -204.1123907548458760 ) ) ;
#52539=CARTESIAN_POINT ( 'NONE',  ( -22.09703248697899980, -279.0465900044581531, -198.5125239602838008 ) ) ;
#52540=CARTESIAN_POINT ( 'NONE',  ( 29.83286993179561719, -277.9938789019153091, -303.8336019008612539 ) ) ;
#52542=CARTESIAN_POINT ( 'NONE',  ( -67.53368684079607931, -273.5001876856134118, -199.5271999569542345 ) ) ;
#52543=CARTESIAN_POINT ( 'NONE',  ( -78.06293712174220900, -293.4202074867801002, -208.0466328765600394 ) ) ;
#52544=FACE_BOUND ( 'NONE', #67699, .T. ) ;
#52546=CARTESIAN_POINT ( 'NONE',  ( 38.42173754026815402, -291.6554605458762808, -267.5071506028702970 ) ) ;
#52547=CARTESIAN_POINT ( 'NONE',  ( 51.70597994816300513, -298.8638448402078893, -197.3452296079273651 ) ) ;
#52549=CARTESIAN_POINT ( 'NONE',  ( -111.3271405602741311, -292.3086944255701951, -251.6305753479940961 ) ) ;
#52550=CARTESIAN_POINT ( 'NONE',  ( 21.27581636871892101, -277.4090924074130839, -223.5744983911110353 ) ) ;
#52551=CARTESIAN_POINT ( 'NONE',  ( 23.46680027001436741, -288.9565606152380610, -226.6578009446622559 ) ) ;
#52552=CARTESIAN_POINT ( 'NONE',  ( 31.96661642615042354, -273.9223669913845356, -298.7191901260448503 ) ) ;
#52553=CARTESIAN_POINT ( 'NONE',  ( 0.1584299730664475991, -276.4756645730788023, -206.0418528563278073 ) ) ;
#52554=CARTESIAN_POINT ( 'NONE',  ( -27.89993318475723783, -290.2526553408465588, -196.4705754324701559 ) ) ;
#52555=CARTESIAN_POINT ( 'NONE',  ( -73.20225697391897768, -281.4423689042412775, -203.6056682192553922 ) ) ;
#52557=CARTESIAN_POINT ( 'NONE',  ( -5.996753444133307021, -281.9775826779881527, -336.4156848240585873 ) ) ;
#52558=CARTESIAN_POINT ( 'NONE',  ( -59.56225951221558290, -278.4130367143945364, -343.7623390193990076 ) ) ;
#52559=CARTESIAN_POINT ( 'NONE',  ( 15.46863383773208156, -281.1200989619532038, -325.8505525105308038 ) ) ;
#52560=CARTESIAN_POINT ( 'NONE',  ( -7.963562319901559050, -277.6178267542222216, -341.2960568440491897 ) ) ;
#52561=CARTESIAN_POINT ( 'NONE',  ( 29.94095155121660312, -277.5429890985238899, -306.4693004799062805 ) ) ;
#52562=CARTESIAN_POINT ( 'NONE',  ( -21.33282851196159058, -291.3376638359844719, -340.3538533559490702 ) ) ;
#52564=CARTESIAN_POINT ( 'NONE',  ( -111.7865451712130493, -298.4300368579363862, -279.8843936647900250 ) ) ;
#52565=CARTESIAN_POINT ( 'NONE',  ( -96.00745841876324960, -291.0170900445153279, -314.3428957959031322 ) ) ;
#52566=CARTESIAN_POINT ( 'NONE',  ( -18.62840938020975301, -274.8300442100257328, -342.6221693801379047 ) ) ;
#52567=CARTESIAN_POINT ( 'NONE',  ( -17.96086906392792315, -290.5657478694196811, -343.8346329294922157 ) ) ;
#52568=CARTESIAN_POINT ( 'NONE',  ( -49.69780222124557412, -291.2391130690448904, -198.2596040534082249 ) ) ;
#52569=CARTESIAN_POINT ( 'NONE',  ( -28.99009523785359121, -288.4567781038294356, -346.8984396358637809 ) ) ;
#52571=CARTESIAN_POINT ( 'NONE',  ( -71.80027827851007771, -281.9154717984976628, -335.6224910033434981 ) ) ;
#52572=CARTESIAN_POINT ( 'NONE',  ( -110.9277180711544730, -292.5446068176033805, -260.1828460679031423 ) ) ;
#52573=CARTESIAN_POINT ( 'NONE',  ( -96.30920432704658651, -283.6466384216956840, -226.1622356147237269 ) ) ;
#52574=CARTESIAN_POINT ( 'NONE',  ( 33.58513878264707131, -282.6141505130743212, -251.0613363609991495 ) ) ;
#52575=CARTESIAN_POINT ( 'NONE',  ( -1.898672013780521750, -289.5355096448350309, -338.4537899210238834 ) ) ;
#52576=CARTESIAN_POINT ( 'NONE',  ( -95.66465954718233888, -279.6623486220472614, -226.3355672370708191 ) ) ;
#52577=CARTESIAN_POINT ( 'NONE',  ( 17.21763306045860986, -291.6041349281219937, -216.5157116783219067 ) ) ;
#52578=CARTESIAN_POINT ( 'NONE',  ( -37.99135895101665739, -286.8470348876525691, -193.5253400875681393 ) ) ;
#52579=CARTESIAN_POINT ( 'NONE',  ( -4.353759592239997644, -289.1213033552859883, -339.8833032786220656 ) ) ;
#52580=CARTESIAN_POINT ( 'NONE',  ( -109.4980266451586886, -284.5685718249876004, -281.7517358723518441 ) ) ;
#52583=CARTESIAN_POINT ( 'NONE',  ( -28.02486418271881163, -294.0294952511274005, -195.1185325640414874 ) ) ;
#52584=CARTESIAN_POINT ( 'NONE',  ( 37.84373358426017830, -292.0587765759620424, -256.2031226685676870 ) ) ;
#52585=CARTESIAN_POINT ( 'NONE',  ( -7.422457413245961533, -275.7086466902309780, -337.2060681591815410 ) ) ;
#52586=CARTESIAN_POINT ( 'NONE',  ( -65.49694695131958611, -297.0422731591007164, -198.7458750182212555 ) ) ;
#52587=CARTESIAN_POINT ( 'NONE',  ( 26.38259440541440526, -292.5350553551820667, -307.3735758496896437 ) ) ;
#52588=CARTESIAN_POINT ( 'NONE',  ( -97.69625947043124370, -295.3820592037396864, -227.5207027046176904 ) ) ;
#52589=CARTESIAN_POINT ( 'NONE',  ( -100.0588241604511381, -292.2794788511437218, -232.2337936940608643 ) ) ;
#52590=CARTESIAN_POINT ( 'NONE',  ( 27.43763179995663037, -295.0986580454518844, -304.7896572345953246 ) ) ;
#52592=CARTESIAN_POINT ( 'NONE',  ( -19.74186261568116407, -292.8263582785700692, -343.4918720160446242 ) ) ;
#52593=CARTESIAN_POINT ( 'NONE',  ( -106.5187409717126457, -298.1724126029107538, -299.4680911956714340 ) ) ;
#52594=CARTESIAN_POINT ( 'NONE',  ( -29.13489213650443332, -289.8868512351302229, -343.1351294874123710 ) ) ;
#52595=CARTESIAN_POINT ( 'NONE',  ( 34.92344219847572617, -277.8063563093791117, -291.7645055544556953 ) ) ;
#52596=CARTESIAN_POINT ( 'NONE',  ( -72.26665628135998531, -278.2847526583374247, -202.2764089129724141 ) ) ;
#52597=CARTESIAN_POINT ( 'NONE',  ( -27.00200147216099111, -273.5287749168124947, -194.1079983406012843 ) ) ;
#52598=CARTESIAN_POINT ( 'NONE',  ( 36.78872309555949016, -279.5371985651728437, -263.0334407236534844 ) ) ;
#52599=CARTESIAN_POINT ( 'NONE',  ( -101.4352498721113136, -276.4045509919511687, -311.6697826534248748 ) ) ;
#52601=CARTESIAN_POINT ( 'NONE',  ( -80.45753435868844861, -294.3352919958117582, -329.8780761990958581 ) ) ;
#52602=CARTESIAN_POINT ( 'NONE',  ( -73.43786540279265296, -275.5738618339977961, -204.5613507086511333 ) ) ;
#52603=CARTESIAN_POINT ( 'NONE',  ( -32.69282475682609856, -274.7636705991545796, -197.3946117842211549 ) ) ;
#52605=CARTESIAN_POINT ( 'NONE',  ( -89.62616398344084701, -289.3399644500694876, -216.0232488371607644 ) ) ;
#52606=CARTESIAN_POINT ( 'NONE',  ( -54.50161534199090596, -289.2666166408383219, -345.4793849556406826 ) ) ;
#52607=CARTESIAN_POINT ( 'NONE',  ( -77.87489449231253502, -275.5091014185332483, -207.0595494411959407 ) ) ;
#52608=CARTESIAN_POINT ( 'NONE',  ( -95.86965410561414558, -295.1944313365081598, -223.7295081601799893 ) ) ;
#52609=CARTESIAN_POINT ( 'NONE',  ( 4.449280717170755572, -281.7013157469030489, -334.9040171347362502 ) ) ;
#52611=CARTESIAN_POINT ( 'NONE',  ( 28.81783187126130485, -280.0219006508491475, -305.7955748485454137 ) ) ;
#52613=CARTESIAN_POINT ( 'NONE',  ( -106.0771239745501475, -289.6903339982882244, -244.4765102920835602 ) ) ;
#52614=CARTESIAN_POINT ( 'NONE',  ( -83.58232285556076135, -281.8333180403552660, -328.5017928378059651 ) ) ;
#52615=CARTESIAN_POINT ( 'NONE',  ( 82.64890176555634582, -299.5541904835127980, -195.3611179825600175 ) ) ;
#52617=CARTESIAN_POINT ( 'NONE',  ( -22.31570140609487396, -290.2444268900834459, -196.8817330632668927 ) ) ;
#52618=CARTESIAN_POINT ( 'NONE',  ( -29.60956401823413486, -278.5528922474309752, -343.8064140483295432 ) ) ;
#52619=CARTESIAN_POINT ( 'NONE',  ( -5.605944055364151524, -283.8490138042897684, -340.0809179424495028 ) ) ;
#52620=CARTESIAN_POINT ( 'NONE',  ( -36.92269341036211472, -272.1372436690941754, -194.7894673150107110 ) ) ;
#52621=CARTESIAN_POINT ( 'NONE',  ( -14.56600449232711014, -286.3556093030103398, -200.9520061194560867 ) ) ;
#52622=CARTESIAN_POINT ( 'NONE',  ( 36.23163741906842006, -276.9574188222558178, -268.8317659534246786 ) ) ;
#52623=CARTESIAN_POINT ( 'NONE',  ( -35.10247309152077122, -277.8261519372910016, -343.4883194173067977 ) ) ;
#52626=CARTESIAN_POINT ( 'NONE',  ( -94.31442759118930041, -287.2286414211441183, -221.5070858983209519 ) ) ;
#52630=CARTESIAN_POINT ( 'NONE',  ( -50.46961047978744119, -295.0485259551674631, -346.2877062656752969 ) ) ;
#52632=CARTESIAN_POINT ( 'NONE',  ( -37.37352853689063181, -292.5523547857346784, -350.3611179825600175 ) ) ;
#52633=CARTESIAN_POINT ( 'NONE',  ( -111.4288308098553273, -277.7221492231461752, -250.4965797437095318 ) ) ;
#52634=CARTESIAN_POINT ( 'NONE',  ( -11.40617662614166683, -290.7842112735534670, -198.6551916763846179 ) ) ;
#52635=CARTESIAN_POINT ( 'NONE',  ( -67.85225702386543389, -287.1643463226504309, -203.2804674777293314 ) ) ;
#52636=CARTESIAN_POINT ( 'NONE',  ( -84.09496531641927675, -281.1598431612854938, -212.9178878779722766 ) ) ;
#52637=CARTESIAN_POINT ( 'NONE',  ( 4.839166937267678215, -288.0347628429412339, -206.5848362945725967 ) ) ;
#52638=CARTESIAN_POINT ( 'NONE',  ( 21.77266947861653890, -284.1855163762223242, -316.5183704909322842 ) ) ;
#52639=CARTESIAN_POINT ( 'NONE',  ( -35.70938148302340664, -277.1989171208280709, -347.3569378957428171 ) ) ;
#52640=CARTESIAN_POINT ( 'NONE',  ( -99.34835060316936506, -271.1211597243290612, -228.3735661696755983 ) ) ;
#52641=CARTESIAN_POINT ( 'NONE',  ( -106.1746257757665290, -278.8307409744800225, -235.7310946939329312 ) ) ;
#52642=CARTESIAN_POINT ( 'NONE',  ( -87.08026348660725091, -299.2731063423513547, -214.9770994351865738 ) ) ;
#52644=CARTESIAN_POINT ( 'NONE',  ( -110.4683760289727132, -275.2662352645559167, -253.7030783399848985 ) ) ;
#52645=CARTESIAN_POINT ( 'NONE',  ( -34.08881529147114975, -296.2320524517635931, -194.5973284279544373 ) ) ;
#52647=CARTESIAN_POINT ( 'NONE',  ( -87.14205353033921142, -277.2765237406758843, -323.8205721748724955 ) ) ;
#52648=CARTESIAN_POINT ( 'NONE',  ( -0.2512162469553667066, -275.7391696561791719, -203.3215459071010116 ) ) ;
#52649=CARTESIAN_POINT ( 'NONE',  ( 4.407645986672851457, -281.5629186366799672, -334.8429746093233348 ) ) ;
#52650=CARTESIAN_POINT ( 'NONE',  ( 16.76688925948248965, -290.0293004739678508, -320.9359810329539187 ) ) ;
#52651=CARTESIAN_POINT ( 'NONE',  ( -103.2607064427807444, -298.5781174793947343, -231.8200814929145110 ) ) ;
#52652=CARTESIAN_POINT ( 'NONE',  ( -102.7684346936857622, -297.2342641213754177, -310.2026932776382750 ) ) ;
#52653=CARTESIAN_POINT ( 'NONE',  ( 35.07609064888190176, -295.3094169972781629, -251.5013192430557467 ) ) ;
#52654=CARTESIAN_POINT ( 'NONE',  ( 36.95692165498365966, -279.6723202598245166, -279.7119766175076165 ) ) ;
#52655=CARTESIAN_POINT ( 'NONE',  ( -6.188666745529876501, -282.3848272374017938, -202.7394928500793014 ) ) ;
#52656=CARTESIAN_POINT ( 'NONE',  ( -55.62412464102188636, -295.8950013746932655, -198.1477697394450956 ) ) ;
#52657=CARTESIAN_POINT ( 'NONE',  ( -82.81497259496194374, -287.0424251864471330, -209.1510349148578882 ) ) ;
#52658=CARTESIAN_POINT ( 'NONE',  ( -5.671286685325179988, -287.5458573154012925, -336.4762523097759868 ) ) ;
#52659=CARTESIAN_POINT ( 'NONE',  ( -29.74821284649360109, -125.1331993717982272, -364.1253139031180694 ) ) ;
#52661=CARTESIAN_POINT ( 'NONE',  ( -45.97734613929616643, -287.7342121783263451, -346.3350604306444325 ) ) ;
#52662=CARTESIAN_POINT ( 'NONE',  ( 35.29586074006135021, -287.1202929560498660, -262.8863445504107403 ) ) ;
#52664=CARTESIAN_POINT ( 'NONE',  ( -41.53841591312731651, -284.1833711727791183, -346.9892107964356569 ) ) ;
#52665=CARTESIAN_POINT ( 'NONE',  ( 15.45914512182664780, -275.1573632520764932, -219.8482788284892990 ) ) ;
#52666=CARTESIAN_POINT ( 'NONE',  ( -94.47181848533857362, -290.1693203314193283, -219.1982204239498628 ) ) ;
#52667=CARTESIAN_POINT ( 'NONE',  ( 37.57630530788240009, -281.9857845721157332, -252.9653204307675196 ) ) ;
#52668=CARTESIAN_POINT ( 'NONE',  ( 10.37423572682743611, -282.2168516784700500, -210.7459696539853553 ) ) ;
#52669=CARTESIAN_POINT ( 'NONE',  ( -21.72613013204149013, -283.1905272761580932, -345.7394853377573440 ) ) ;
#52670=CARTESIAN_POINT ( 'NONE',  ( -89.47357884723847121, -279.2925092449667659, -219.1889198564007302 ) ) ;
#52671=CARTESIAN_POINT ( 'NONE',  ( -20.19161114001082069, -277.7666405000204009, -195.3683826091709363 ) ) ;
#52672=CARTESIAN_POINT ( 'NONE',  ( 204.1737866480590924, 295.5637011240619927, -68.68209524862845683 ) ) ;
#52674=CARTESIAN_POINT ( 'NONE',  ( 34.61601920761162177, -277.2851623686695461, -249.6307470447542016 ) ) ;
#52675=CARTESIAN_POINT ( 'NONE',  ( -22.99186949233678945, -107.8477965757182204, -362.2362941995334040 ) ) ;
#52676=CARTESIAN_POINT ( 'NONE',  ( -52.64834823549384168, -297.1995538209649226, -198.8277007655893556 ) ) ;
#52677=CARTESIAN_POINT ( 'NONE',  ( 37.36369790267395530, -292.8294194253056730, -251.9592048057795353 ) ) ;
#52678=CARTESIAN_POINT ( 'NONE',  ( 193.8404912568037446, 275.6304219183343207, -124.1201750202075687 ) ) ;
#52679=CARTESIAN_POINT ( 'NONE',  ( -77.87441223988015793, -296.0936238627925832, -205.5868519423754321 ) ) ;
#52680=CARTESIAN_POINT ( 'NONE',  ( -37.28766759898142169, -287.4513352148392187, -344.1611010333646732 ) ) ;
#52681=CARTESIAN_POINT ( 'NONE',  ( -50.67011203268599218, -297.0846205352576135, -343.3900089355659020 ) ) ;
#52682=CARTESIAN_POINT ( 'NONE',  ( -74.98700277213917786, -286.8544849772890757, -207.2415911555131061 ) ) ;
#52684=CARTESIAN_POINT ( 'NONE',  ( -64.17268463485460472, -296.3350648556469764, -342.2841218353725026 ) ) ;
#52685=CARTESIAN_POINT ( 'NONE',  ( -110.2900917439872615, -285.1090053368810686, -265.4673239033900245 ) ) ;
#52686=CARTESIAN_POINT ( 'NONE',  ( -26.26561591906065729, -296.9828540441263840, -193.7603967612039924 ) ) ;
#52687=CARTESIAN_POINT ( 'NONE',  ( -68.27316159071216362, -292.4589576487653630, -200.0089986674241800 ) ) ;
#52688=CARTESIAN_POINT ( 'NONE',  ( 19.36606221550634999, -293.3364986157773160, -218.3634584847602014 ) ) ;
#52689=CARTESIAN_POINT ( 'NONE',  ( -50.74938228436087684, -289.3947620357002961, -342.1709602780546788 ) ) ;
#52692=CARTESIAN_POINT ( 'NONE',  ( -36.23122460170400672, -299.9263225365933181, -194.5959630375046743 ) ) ;
#52693=CARTESIAN_POINT ( 'NONE',  ( -32.69129527004988489, -272.9044345745654141, -193.8863948477479369 ) ) ;
#52697=CARTESIAN_POINT ( 'NONE',  ( 27.59352157778364401, -275.6022134199692459, -311.7268783411288950 ) ) ;
#52699=CARTESIAN_POINT ( 'NONE',  ( -54.37663549347558956, -272.2295192979731269, -198.5540752214207032 ) ) ;
#52700=CARTESIAN_POINT ( 'NONE',  ( -107.4225647998200373, -280.0904514913161734, -295.0023346710380565 ) ) ;
#52701=CARTESIAN_POINT ( 'NONE',  ( -7.024518934781800006, -274.7896313874917382, -338.1234527071920297 ) ) ;
#52702=CARTESIAN_POINT ( 'NONE',  ( -84.34080488233216499, -298.5939842164213474, -213.9190915884640560 ) ) ;
#52703=CARTESIAN_POINT ( 'NONE',  ( -63.40161717392884810, -274.6453448481150872, -201.9057128947075341 ) ) ;
#52704=CARTESIAN_POINT ( 'NONE',  ( -32.00007760669642920, -299.7180926278506945, -194.1596863099827885 ) ) ;
#52705=CARTESIAN_POINT ( 'NONE',  ( 22.34581165502161326, -272.9447924783620465, -224.3421961973749319 ) ) ;
#52706=CARTESIAN_POINT ( 'NONE',  ( 34.81321736065179095, -294.0480334721162876, -258.5542756019498825 ) ) ;
#52707=CARTESIAN_POINT ( 'NONE',  ( -41.60900291774942872, -290.5722191460443469, -196.8454682842868237 ) ) ;
#52709=CARTESIAN_POINT ( 'NONE',  ( -39.95457795819446289, -277.5764680703449585, -347.2682553160324233 ) ) ;
#52710=CARTESIAN_POINT ( 'NONE',  ( 35.35420273350267450, -275.8066402417032918, -277.0173715558327672 ) ) ;
#52712=CARTESIAN_POINT ( 'NONE',  ( -106.2277704425618197, -283.6668320181299237, -237.0743700481887402 ) ) ;
#52713=CARTESIAN_POINT ( 'NONE',  ( 20.88308640062745170, -296.2061393548696628, -317.9197665947267524 ) ) ;
#52715=CARTESIAN_POINT ( 'NONE',  ( -89.77145539793603746, -284.4862672667557035, -219.2617449393218578 ) ) ;
#52716=CARTESIAN_POINT ( 'NONE',  ( -110.7405302030631589, -282.3443717192058102, -286.5672950407857797 ) ) ;
#52717=CARTESIAN_POINT ( 'NONE',  ( -41.94165185004501950, -275.3507339666684288, -344.2441434208323585 ) ) ;
#52718=CARTESIAN_POINT ( 'NONE',  ( -7.283448734543601866, -275.2247046621117192, -337.5316207478356318 ) ) ;
#52719=CARTESIAN_POINT ( 'NONE',  ( 36.55104501111865289, -283.3865060799023468, -257.4477512657309148 ) ) ;
#52720=CARTESIAN_POINT ( 'NONE',  ( 33.63004823419364442, -277.0029778877860167, -289.0731846822382067 ) ) ;
#52722=CARTESIAN_POINT ( 'NONE',  ( -46.76169259700797198, -272.3343199022644399, -194.7456158935853807 ) ) ;
#52723=CARTESIAN_POINT ( 'NONE',  ( -34.02234085966953359, -282.0939795260514416, -195.2677741847248285 ) ) ;
#52725=CARTESIAN_POINT ( 'NONE',  ( 6.684667905823711287, -288.5653779333867419, -208.8882781638876907 ) ) ;
#52727=CARTESIAN_POINT ( 'NONE',  ( -108.8813797260759486, -288.2595266195689305, -293.0472744037678581 ) ) ;
#52729=CARTESIAN_POINT ( 'NONE',  ( -108.6886094718227866, -295.1203636427646302, -287.6405681808222425 ) ) ;
#52730=CARTESIAN_POINT ( 'NONE',  ( -111.5420422543510170, -288.6452337711638165, -273.9453638151793484 ) ) ;
#52731=CARTESIAN_POINT ( 'NONE',  ( 201.7648208617462728, 289.3015991269851384, -82.29596988341933184 ) ) ;
#52733=CARTESIAN_POINT ( 'NONE',  ( -3.386799957615262535, -287.0919661782725143, -338.7113471063460111 ) ) ;
#52734=CARTESIAN_POINT ( 'NONE',  ( 18.22044941193164647, -283.8377616127854139, -318.9336200276972022 ) ) ;
#52735=CARTESIAN_POINT ( 'NONE',  ( -104.8937111162223346, -282.3362796204760343, -305.2711007055088430 ) ) ;
#52736=CARTESIAN_POINT ( 'NONE',  ( -89.81632044842253038, -291.2854897873501159, -219.6125788682560938 ) ) ;
#52737=CARTESIAN_POINT ( 'NONE',  ( 24.16511653705481777, -282.4206611920876639, -229.8676902555195625 ) ) ;
#52738=CARTESIAN_POINT ( 'NONE',  ( 30.48805397941071504, -282.7213310520731966, -297.7787434135553326 ) ) ;
#52739=CARTESIAN_POINT ( 'NONE',  ( -109.2054530565073520, -292.2389411195912317, -293.2031420081622741 ) ) ;
#52741=CARTESIAN_POINT ( 'NONE',  ( -37.60979226633180872, -298.2155611169161489, -193.3615846648643810 ) ) ;
#52743=CARTESIAN_POINT ( 'NONE',  ( -67.50198497119713181, -287.5245596067173324, -339.6407789118019309 ) ) ;
#52744=CARTESIAN_POINT ( 'NONE',  ( 37.28522715503766705, -275.3147902972951897, -251.3921505810363044 ) ) ;
#52745=CARTESIAN_POINT ( 'NONE',  ( -58.13681119472654757, -293.7621706632082805, -198.6173647044027746 ) ) ;
#52747=CARTESIAN_POINT ( 'NONE',  ( -4.829096099716510437, -282.9805209788416391, -202.7746430608542312 ) ) ;
#52748=CARTESIAN_POINT ( 'NONE',  ( -42.70148299504471368, -275.1194821086073148, -345.3364549598027224 ) ) ;
#52750=CARTESIAN_POINT ( 'NONE',  ( -110.0436413100536441, -295.2438037109412221, -247.3638211004543734 ) ) ;
#52751=CARTESIAN_POINT ( 'NONE',  ( -82.23163505869359824, -293.0285670518632628, -211.7188467496689839 ) ) ;
#52752=CARTESIAN_POINT ( 'NONE',  ( 11.62094243344143685, -274.1014709532460643, -216.0107967717650581 ) ) ;
#52753=CARTESIAN_POINT ( 'NONE',  ( -109.3359468303453639, -291.8659714999176913, -286.1529908743489727 ) ) ;
#52754=CARTESIAN_POINT ( 'NONE',  ( -30.79784705659721311, -293.0781552111933479, -197.4187679031359721 ) ) ;
#52755=CARTESIAN_POINT ( 'NONE',  ( -88.40966833911096501, -287.0845522022424348, -216.7883951211339024 ) ) ;
#52757=CARTESIAN_POINT ( 'NONE',  ( 21.74201416361712447, -294.3217109682483397, -221.9078311938118588 ) ) ;
#52758=CARTESIAN_POINT ( 'NONE',  ( -25.11684727967028863, -293.5200938648910665, -194.8372724470382593 ) ) ;
#52759=CARTESIAN_POINT ( 'NONE',  ( 19.69243349044737101, -294.0293084894926210, -315.9453681172162192 ) ) ;
#52760=CARTESIAN_POINT ( 'NONE',  ( 35.32004266666400127, -289.3129832617185002, -251.7278616859402405 ) ) ;
#52761=CARTESIAN_POINT ( 'NONE',  ( 38.14596882137117007, -281.9087520919610483, -285.5470272772021190 ) ) ;
#52762=CARTESIAN_POINT ( 'NONE',  ( -108.0058485851963610, -271.0452241381656791, -242.8876531527655800 ) ) ;
#52763=CARTESIAN_POINT ( 'NONE',  ( -91.90149400844251204, -285.1328143694960886, -216.0267007478929600 ) ) ;
#52764=CARTESIAN_POINT ( 'NONE',  ( 37.28684134950955098, -277.5119494470968675, -268.8030433531653216 ) ) ;
#52766=CARTESIAN_POINT ( 'NONE',  ( -97.67363213449614534, -283.9265649402213398, -228.5395246498943891 ) ) ;
#52768=CARTESIAN_POINT ( 'NONE',  ( 24.71716566015151884, -284.9816810456520670, -228.2228731065362695 ) ) ;
#52769=CARTESIAN_POINT ( 'NONE',  ( -71.92157598159991494, -277.7395989226884012, -202.9335173445587088 ) ) ;
#52771=CARTESIAN_POINT ( 'NONE',  ( -73.83296191148022558, -283.0580651437806523, -333.7147145270577653 ) ) ;
#52772=CARTESIAN_POINT ( 'NONE',  ( -112.8477081509243760, -279.9196071709312719, -257.4440180173717749 ) ) ;
#52773=CARTESIAN_POINT ( 'NONE',  ( 35.72012185478266133, -286.9080193733327064, -293.9151066341677279 ) ) ;
#52774=CARTESIAN_POINT ( 'NONE',  ( -34.23655326212983852, -296.7727192773767229, -344.3092895495694279 ) ) ;
#52775=CARTESIAN_POINT ( 'NONE',  ( -4.322871206772958885, -278.2243319901469363, -339.0500441296923668 ) ) ;
#52776=CARTESIAN_POINT ( 'NONE',  ( -88.86755277788768126, -279.0734126108891928, -326.9153820160118471 ) ) ;
#52777=CARTESIAN_POINT ( 'NONE',  ( -109.9658807617877017, -278.4894505899445107, -262.4789091549683349 ) ) ;
#52778=CARTESIAN_POINT ( 'NONE',  ( -97.59114340725315628, -299.1593410089073473, -225.9544209299175463 ) ) ;
#52779=CARTESIAN_POINT ( 'NONE',  ( 36.77263327021314154, -285.6863584788189883, -280.8028135161503087 ) ) ;
#52780=CARTESIAN_POINT ( 'NONE',  ( -45.91530714428242987, -290.7591252826912296, -346.1298310116757193 ) ) ;
#52782=CARTESIAN_POINT ( 'NONE',  ( -41.06862874634942528, -294.0204468436998582, -343.5880544860913233 ) ) ;
#52784=CARTESIAN_POINT ( 'NONE',  ( 33.46552525166386260, -293.4543078974760419, -288.2055658832317135 ) ) ;
#52786=CARTESIAN_POINT ( 'NONE',  ( -12.31157078130881288, -289.8138243848017055, -342.9080456449955250 ) ) ;
#52787=CARTESIAN_POINT ( 'NONE',  ( -64.86217238904167459, -280.3343581237639910, -202.6372944427344578 ) ) ;
#52788=CARTESIAN_POINT ( 'NONE',  ( -85.01348543588264306, -296.3319389294528605, -210.2870520769135680 ) ) ;
#52789=CARTESIAN_POINT ( 'NONE',  ( 31.32704074539721617, -287.7575967804397123, -235.7501831046484426 ) ) ;
#52790=CARTESIAN_POINT ( 'NONE',  ( -78.12160448586301698, -289.9174123739140327, -335.7129868138432585 ) ) ;
#52791=CARTESIAN_POINT ( 'NONE',  ( -108.4449147762774572, -284.6655195997381611, -287.0416297760234556 ) ) ;
#52792=DIRECTION ( 'NONE',  ( 1.000000000000000000, 0.000000000000000000, 0.000000000000000000 ) ) ;
#52793=CARTESIAN_POINT ( 'NONE',  ( 159.4317074227722912, 220.1917126582878268, -204.0458204816173691 ) ) ;
#52794=CARTESIAN_POINT ( 'NONE',  ( -39.68813811115344947, -139.7239799056983998, -360.9171517653596197 ) ) ;
#52795=CARTESIAN_POINT ( 'NONE',  ( -85.21861693474863841, -276.9303143095906421, -325.7491400160296280 ) ) ;
#52796=CARTESIAN_POINT ( 'NONE',  ( -109.9258838242978982, -277.6121890963433998, -259.7252640482822699 ) ) ;
#52797=CARTESIAN_POINT ( 'NONE',  ( -55.32456115304022148, -273.4936205805251461, -195.5121968093566238 ) ) ;
#52798=CARTESIAN_POINT ( 'NONE',  ( -104.5539746777214702, -261.5182135941884098, -316.0123334579292873 ) ) ;
#52799=CARTESIAN_POINT ( 'NONE',  ( -77.56993866038361318, -276.2645236304657601, -335.4994676586070455 ) ) ;
#52801=CARTESIAN_POINT ( 'NONE',  ( -109.8498178543374593, -290.9261986689280661, -279.3367129728978853 ) ) ;
#52802=CARTESIAN_POINT ( 'NONE',  ( -14.87906221710319521, -299.1295042059245475, -193.5196183270483061 ) ) ;
#52803=CARTESIAN_POINT ( 'NONE',  ( 28.66337167796363516, -286.6718405963765122, -302.6809876054566075 ) ) ;
#52804=CARTESIAN_POINT ( 'NONE',  ( -113.4446582428203101, -273.3462381016220206, -258.9680425074045047 ) ) ;
#52805=CARTESIAN_POINT ( 'NONE',  ( -107.9690378533114625, -296.4745153769831063, -288.8707401918701407 ) ) ;
#52808=CARTESIAN_POINT ( 'NONE',  ( -77.03719570818101658, -279.4993301686889140, -334.7148469967547726 ) ) ;
#52809=CARTESIAN_POINT ( 'NONE',  ( 32.33399618368085982, -281.4793906983199463, -303.1182592167069174 ) ) ;
#52810=CARTESIAN_POINT ( 'NONE',  ( -110.5884271342985272, -279.5921097571983296, -273.3848665844764128 ) ) ;
#52811=CARTESIAN_POINT ( 'NONE',  ( -110.7578647047998857, -280.5615028494339640, -250.7138682111082062 ) ) ;
#52812=CARTESIAN_POINT ( 'NONE',  ( -99.85852029930474316, -271.5655069418538119, -231.3437507282046681 ) ) ;
#52814=CARTESIAN_POINT ( 'NONE',  ( -30.26449800094154696, -280.3107140210297530, -197.6546329628944818 ) ) ;
#52815=CARTESIAN_POINT ( 'NONE',  ( -2.788545181048796007, -277.4099544044010486, -339.0069418778946897 ) ) ;
#52816=CARTESIAN_POINT ( 'NONE',  ( 24.48114636701398794, -276.9766916701054242, -227.8773682684846165 ) ) ;
#52817=CARTESIAN_POINT ( 'NONE',  ( -8.126841969556080514, -275.2516846503793886, -340.9805206333419960 ) ) ;
#52820=CARTESIAN_POINT ( 'NONE',  ( -106.7211857637723114, -290.0570064304056359, -247.1428342424025857 ) ) ;
#52821=CARTESIAN_POINT ( 'NONE',  ( -35.14282849889130489, -285.4276391690336254, -193.4813689071053773 ) ) ;
#52822=CARTESIAN_POINT ( 'NONE',  ( -110.8822364370469700, -282.6775636605867135, -279.1568319559953579 ) ) ;
#52824=CARTESIAN_POINT ( 'NONE',  ( -7.027200495402667890, -281.2211402287438204, -337.4301864915074702 ) ) ;
#52825=CARTESIAN_POINT ( 'NONE',  ( -19.44646104965246991, -284.3639727740243188, -198.1041140780924650 ) ) ;
#52827=CARTESIAN_POINT ( 'NONE',  ( 25.22149642160500704, -290.1119102845617022, -311.8161132101660655 ) ) ;
#52828=CARTESIAN_POINT ( 'NONE',  ( -22.12699886173711050, -281.4563536819765659, -198.5061716987787008 ) ) ;
#52829=CARTESIAN_POINT ( 'NONE',  ( -111.8722755992515800, -270.6595642643046631, -261.9829339559319692 ) ) ;
#52830=CARTESIAN_POINT ( 'NONE',  ( 30.35697287138012967, -280.4076286439792511, -305.3372539550782108 ) ) ;
#52831=CARTESIAN_POINT ( 'NONE',  ( 16.15335719093937072, -296.2938587509344188, -323.0019167985424247 ) ) ;
#52832=CARTESIAN_POINT ( 'NONE',  ( -94.18861208088614489, -277.4843187276652543, -219.9388747130817023 ) ) ;
#52834=CARTESIAN_POINT ( 'NONE',  ( -72.88431817205568564, -278.1877008478857647, -334.2552104160218391 ) ) ;
#52835=CARTESIAN_POINT ( 'NONE',  ( -37.99274674150289854, -288.0441689586845087, -195.1972665018789996 ) ) ;
#52837=CARTESIAN_POINT ( 'NONE',  ( -70.29226251824722738, -293.5414334964053751, -202.3642456944826620 ) ) ;
#52838=CARTESIAN_POINT ( 'NONE',  ( 35.16948615312456639, -273.7982598852104843, -289.5217159807754683 ) ) ;
#52839=CARTESIAN_POINT ( 'NONE',  ( -73.10779325498795345, -288.7111114407824743, -338.3827954629169881 ) ) ;
#52840=CARTESIAN_POINT ( 'NONE',  ( -14.58052054456640079, -290.7520197055860081, -200.1587738769403018 ) ) ;
#52842=CARTESIAN_POINT ( 'NONE',  ( -74.27549655622148350, -276.2391080209486631, -333.8995957708779088 ) ) ;
#52843=CARTESIAN_POINT ( 'NONE',  ( -99.78492158301806114, -294.1443065307786355, -310.6014342814366387 ) ) ;
#52844=CARTESIAN_POINT ( 'NONE',  ( -109.4191141173435824, -291.6783802566276904, -284.7812456618848955 ) ) ;
#52847=CARTESIAN_POINT ( 'NONE',  ( 36.04275873721073964, -291.7669403933651893, -249.3986615262905104 ) ) ;
#52848=CARTESIAN_POINT ( 'NONE',  ( 27.05560708662114777, -288.6632888032719393, -234.2090409928904648 ) ) ;
#52849=CARTESIAN_POINT ( 'NONE',  ( -101.4584337724489416, -288.2492599616738289, -311.2381121573827158 ) ) ;
#52850=CARTESIAN_POINT ( 'NONE',  ( 26.87274919344519475, -288.4884608640265355, -234.3141791509244740 ) ) ;
#52852=CARTESIAN_POINT ( 'NONE',  ( 31.12209605237864096, -288.0098328072009508, -244.4245517556633160 ) ) ;
#52853=CARTESIAN_POINT ( 'NONE',  ( -58.36767796827526666, -297.3023644872446312, -342.7778845247910340 ) ) ;
#52855=CARTESIAN_POINT ( 'NONE',  ( 37.44067781889307156, -288.9666742209906261, -287.0224002332747091 ) ) ;
#52856=CARTESIAN_POINT ( 'NONE',  ( -34.37262320475240074, -275.0949447357804729, -345.8627655304486552 ) ) ;
#52857=CARTESIAN_POINT ( 'NONE',  ( -111.4190136797459445, -278.6229744271665822, -291.2966358536714324 ) ) ;
#52858=CARTESIAN_POINT ( 'NONE',  ( -93.05551746675897107, -278.9460170913204138, -217.1651463320342543 ) ) ;
#52859=CARTESIAN_POINT ( 'NONE',  ( -97.43923713673152065, -299.1390759897273597, -226.0661418624069938 ) ) ;
#52860=CARTESIAN_POINT ( 'NONE',  ( -96.51986230846380010, -283.1841407724330679, -224.2648371492523438 ) ) ;
#52862=CARTESIAN_POINT ( 'NONE',  ( -27.36937928137762555, -278.3196412620700926, -196.7467161590899991 ) ) ;
#52863=CARTESIAN_POINT ( 'NONE',  ( -70.86816973665412434, -281.4943253534577821, -337.4504352275245083 ) ) ;
#52865=CARTESIAN_POINT ( 'NONE',  ( -3.054153816885291750, -275.0873756752500299, -338.5450976772041827 ) ) ;
#52866=CARTESIAN_POINT ( 'NONE',  ( -97.74064010755812149, -297.4890610725284432, -312.5828635937504600 ) ) ;
#52867=CARTESIAN_POINT ( 'NONE',  ( -71.61299339516558859, -282.4146654591520473, -338.9684861646819058 ) ) ;
#52868=CARTESIAN_POINT ( 'NONE',  ( -107.6887101570641079, -297.7618895802689281, -249.9967709899610497 ) ) ;
#52869=CARTESIAN_POINT ( 'NONE',  ( -26.31508129919702554, -299.5026522738583026, -193.8518589591636783 ) ) ;
#52870=CARTESIAN_POINT ( 'NONE',  ( -14.05468214643588887, -274.0294635639677949, -201.1527205133580480 ) ) ;
#52871=CARTESIAN_POINT ( 'NONE',  ( 30.53809882329510472, -295.1315086098708207, -238.3429694970579931 ) ) ;
#52872=CARTESIAN_POINT ( 'NONE',  ( 28.90482438819904232, -288.2301685438775394, -309.6090223088555717 ) ) ;
#52873=CARTESIAN_POINT ( 'NONE',  ( -103.5203790401297823, -277.1133310609986324, -233.8961121139607826 ) ) ;
#52874=CARTESIAN_POINT ( 'NONE',  ( -97.29141447937213627, -289.7374861096076302, -318.7040782949550248 ) ) ;
#52875=CARTESIAN_POINT ( 'NONE',  ( -100.5129623374312757, -289.1025978490149555, -307.5123437947870002 ) ) ;
#52876=CARTESIAN_POINT ( 'NONE',  ( 34.38200405421400774, -291.2693564601977414, -248.4359975098352891 ) ) ;
#52879=CARTESIAN_POINT ( 'NONE',  ( -104.1065005738800266, -289.6591952903842753, -300.1584588779952014 ) ) ;
#52881=CARTESIAN_POINT ( 'NONE',  ( -65.15572444676007535, -284.3480930052128883, -341.9238641087768542 ) ) ;
#52882=CARTESIAN_POINT ( 'NONE',  ( 39.26644811233330756, -292.6820633193152617, -276.0337351328423097 ) ) ;
#52883=CARTESIAN_POINT ( 'NONE',  ( 37.66539852573927050, -283.0570603285356128, -285.4353816718631833 ) ) ;
#52884=CARTESIAN_POINT ( 'NONE',  ( -1.253852617203371267, -282.3923338942843770, -333.8171442254862313 ) ) ;
#52885=CARTESIAN_POINT ( 'NONE',  ( -80.62502170165275572, -297.4831521112486143, -206.6137783220986250 ) ) ;
#52886=CARTESIAN_POINT ( 'NONE',  ( 21.24008799144644399, -277.4867559308806335, -314.7392384929083846 ) ) ;
#52887=CARTESIAN_POINT ( 'NONE',  ( 30.23813378314736866, -291.1520963426760886, -238.5402586313514917 ) ) ;
#52888=CARTESIAN_POINT ( 'NONE',  ( -16.51336718030072959, -273.1221465266997370, -199.9283559951378493 ) ) ;
#52892=CARTESIAN_POINT ( 'NONE',  ( -24.92523695310635645, -288.1317618822296254, -196.9116328052222400 ) ) ;
#52893=CARTESIAN_POINT ( 'NONE',  ( -96.26505957714701367, -296.9686803682694176, -319.4684986374722371 ) ) ;
#52894=CARTESIAN_POINT ( 'NONE',  ( -107.8572869369304783, -284.9487349115707957, -289.6812583194907802 ) ) ;
#52895=CARTESIAN_POINT ( 'NONE',  ( -68.92954192339310282, -276.5161724624428530, -340.3399598094454745 ) ) ;
#52896=CARTESIAN_POINT ( 'NONE',  ( 37.00015142589705164, -294.4500412056358982, -290.0233125297866081 ) ) ;
#52897=CARTESIAN_POINT ( 'NONE',  ( 31.72894637059891920, -286.0959716072634933, -301.4987362296672586 ) ) ;
#52899=CARTESIAN_POINT ( 'NONE',  ( 33.39881656458503301, -294.2737037300373686, -300.8523605945501345 ) ) ;
#52900=CARTESIAN_POINT ( 'NONE',  ( -83.84576561169004094, -291.7259993838657124, -214.0631661532510179 ) ) ;
#52903=CARTESIAN_POINT ( 'NONE',  ( -109.4300717440927997, -269.0112169713434582, -295.3470023912169609 ) ) ;
#52905=CARTESIAN_POINT ( 'NONE',  ( -110.8185765141799664, -285.8119414575437531, -290.9488908156019420 ) ) ;
#52906=CARTESIAN_POINT ( 'NONE',  ( -69.91165696735023971, -292.9809262143061801, -337.9199732462171255 ) ) ;
#52908=CARTESIAN_POINT ( 'NONE',  ( -51.08928946488654788, -282.1521856814465536, -342.4214544691175206 ) ) ;
#52909=CARTESIAN_POINT ( 'NONE',  ( -114.1894973160493834, -278.2750411820364889, -265.8710891626689090 ) ) ;
#52910=CARTESIAN_POINT ( 'NONE',  ( 26.69217992362646186, -283.0311184695250404, -231.5349147641474872 ) ) ;
#52911=CARTESIAN_POINT ( 'NONE',  ( 186.9921997741134874, 261.2987433936410753, -152.4087338747540343 ) ) ;
#52912=CARTESIAN_POINT ( 'NONE',  ( -41.55494075974604584, -281.6788319875972775, -346.7075708460292276 ) ) ;
#52913=CARTESIAN_POINT ( 'NONE',  ( 37.27298318533834021, -285.6174132796443246, -273.8615511421464248 ) ) ;
#52914=CARTESIAN_POINT ( 'NONE',  ( 15.15386417747978065, -276.6441548003469961, -215.7303463689980276 ) ) ;
#52915=CARTESIAN_POINT ( 'NONE',  ( -41.03606502414044144, -295.5922114829648990, -343.3417718623419432 ) ) ;
#52916=CARTESIAN_POINT ( 'NONE',  ( -7.051796838840049375, -291.1429634180491917, -203.4001947657375524 ) ) ;
#52917=CARTESIAN_POINT ( 'NONE',  ( -113.1374199070956337, -279.3660340736049079, -257.3872346043302741 ) ) ;
#52918=CARTESIAN_POINT ( 'NONE',  ( -45.90809833673234408, -277.1636558391409721, -342.9073768484916513 ) ) ;
#52919=CARTESIAN_POINT ( 'NONE',  ( -91.95860984523744719, -274.3742695399199647, -216.5235318333530188 ) ) ;
#52920=CARTESIAN_POINT ( 'NONE',  ( -62.31836764008141927, -276.2897727279634523, -342.9269177751296525 ) ) ;
#52921=CARTESIAN_POINT ( 'NONE',  ( -114.1313572138536756, -273.4603215278654034, -270.3726811538930406 ) ) ;
#52922=CARTESIAN_POINT ( 'NONE',  ( -71.10962066431646633, -275.4976060606911688, -337.3433636945234184 ) ) ;
#52923=CARTESIAN_POINT ( 'NONE',  ( 13.02120570071824801, -295.7904190895197303, -327.8959196409172705 ) ) ;
#52926=CARTESIAN_POINT ( 'NONE',  ( -110.5377808231913264, -285.6962349906131635, -265.4581718816438070 ) ) ;
#52927=CARTESIAN_POINT ( 'NONE',  ( -107.2855023687954343, -285.9277146292558314, -300.1913977338916766 ) ) ;
#52928=CARTESIAN_POINT ( 'NONE',  ( 25.04202366807640701, -286.3764446069573637, -232.2538526206583356 ) ) ;
#52929=CARTESIAN_POINT ( 'NONE',  ( -67.14420636782639917, -275.8494032447125051, -337.8759388639248300 ) ) ;
#52930=CARTESIAN_POINT ( 'NONE',  ( 27.95254771904341240, -283.8864505880648039, -305.6814616368637871 ) ) ;
#52931=CARTESIAN_POINT ( 'NONE',  ( -26.94262829620306121, -275.3973957843101630, -343.3170434189988214 ) ) ;
#52933=CARTESIAN_POINT ( 'NONE',  ( -59.27443785015729816, -278.4225302841888947, -340.3123945185845400 ) ) ;
#52936=CARTESIAN_POINT ( 'NONE',  ( -65.84292934857880653, -274.1612808213567405, -203.0880299406145753 ) ) ;
#52937=CARTESIAN_POINT ( 'NONE',  ( -1.220403248673440633, -281.3218338926274100, -202.5421624273162706 ) ) ;
#52938=CARTESIAN_POINT ( 'NONE',  ( -19.77637039212308778, -280.7643475223692349, -195.3998767140380721 ) ) ;
#52940=ORIENTED_EDGE ( 'NONE', *, *, #37043, .F. ) ;
#52942=CARTESIAN_POINT ( 'NONE',  ( 37.56078752127080378, -289.2665936233599382, -258.8765448690845687 ) ) ;
#52943=CARTESIAN_POINT ( 'NONE',  ( -110.5458421655025631, -295.7349115658649339, -271.4553519522693819 ) ) ;
#52944=CARTESIAN_POINT ( 'NONE',  ( -92.73289361938923037, -290.6326221338760547, -216.9456264775200225 ) ) ;
#52945=CARTESIAN_POINT ( 'NONE',  ( 35.20081947324865723, -286.2015476355265378, -283.3338048062519192 ) ) ;
#52946=CARTESIAN_POINT ( 'NONE',  ( -15.69551543743928690, -287.3413870195105915, -340.7479812429321555 ) ) ;
#52947=CARTESIAN_POINT ( 'NONE',  ( -27.80004502404392142, -287.3811029544205553, -197.5868964331813231 ) ) ;
#52948=CARTESIAN_POINT ( 'NONE',  ( -68.21596190209044153, -275.4574352439856852, -338.7255761431582641 ) ) ;
#52949=CARTESIAN_POINT ( 'NONE',  ( 30.96119841013293694, -286.3920612148663167, -304.2610323384864728 ) ) ;
#52950=CARTESIAN_POINT ( 'NONE',  ( -67.71477923858087422, -287.6537837843613374, -201.7725056304563509 ) ) ;
#52951=CARTESIAN_POINT ( 'NONE',  ( -10.24848132093128683, -286.6991876887565809, -340.4752101572107108 ) ) ;
#52952=CARTESIAN_POINT ( 'NONE',  ( -59.00633739944922240, -284.2805763211763974, -340.3719291050030051 ) ) ;
#52953=CARTESIAN_POINT ( 'NONE',  ( -85.36186015661988336, -293.3909304980733737, -212.4653850451964843 ) ) ;
#52954=CARTESIAN_POINT ( 'NONE',  ( 82.15278769198762632, -299.2458075654235472, -193.3794153738201942 ) ) ;
#52956=CARTESIAN_POINT ( 'NONE',  ( -105.2304370271346556, -298.9063830277762008, -237.1883339964281276 ) ) ;
#52958=CARTESIAN_POINT ( 'NONE',  ( -24.83876581564859265, -279.4129113542517189, -198.2759020219323247 ) ) ;
#52959=CARTESIAN_POINT ( 'NONE',  ( 23.41763057008242654, -280.1509791256234507, -314.3524546316896817 ) ) ;
#52960=CARTESIAN_POINT ( 'NONE',  ( -32.03389183627948000, -294.1839943711370893, -347.0293249437656300 ) ) ;
#52961=CARTESIAN_POINT ( 'NONE',  ( -111.1983153317845705, -270.8641581079432967, -264.8155075547770139 ) ) ;
#52962=CARTESIAN_POINT ( 'NONE',  ( 36.81500955481342174, -273.5407523786277011, -263.3081620640912206 ) ) ;
#52963=CARTESIAN_POINT ( 'NONE',  ( -50.54346519758605893, -296.5394663848581445, -342.6588141822074931 ) ) ;
#52965=CARTESIAN_POINT ( 'NONE',  ( -113.7524713807139847, -271.1271092548682873, -270.3430111821825790 ) ) ;
#52966=CARTESIAN_POINT ( 'NONE',  ( -69.12476854696672035, -293.7043150738253985, -339.3957269854918195 ) ) ;
#52967=CARTESIAN_POINT ( 'NONE',  ( 30.39103089515177558, -294.5927094717742989, -241.4618840749325841 ) ) ;
#52969=CARTESIAN_POINT ( 'NONE',  ( 13.00689367574113398, -293.5803556918614277, -217.2798517143304764 ) ) ;
#52973=CARTESIAN_POINT ( 'NONE',  ( -32.38879771034004307, -284.1343958998429571, -195.1559757263966617 ) ) ;
#52974=CARTESIAN_POINT ( 'NONE',  ( -42.38972445051935978, -295.1175873543253942, -343.1863708172744509 ) ) ;
#52975=CARTESIAN_POINT ( 'NONE',  ( -31.63628840493104022, -282.9820349885084170, -347.1627201842926524 ) ) ;
#52976=CARTESIAN_POINT ( 'NONE',  ( 38.26933019700478411, -283.4666088895169196, -269.9139198983525603 ) ) ;
#52978=CARTESIAN_POINT ( 'NONE',  ( -32.30356362843286888, -285.7807410796282852, -193.5341449109557175 ) ) ;
#52979=CARTESIAN_POINT ( 'NONE',  ( -84.97693536769345712, -289.3929332568648078, -212.6470574160508136 ) ) ;
#52980=CARTESIAN_POINT ( 'NONE',  ( 13.20688177674606045, -280.8407585787695666, -327.5939101614723086 ) ) ;
#52982=CARTESIAN_POINT ( 'NONE',  ( 5.023221169071004688, -285.3227047679677071, -210.2450494071990192 ) ) ;
#52983=CARTESIAN_POINT ( 'NONE',  ( -23.38175571388271123, -287.7981557650520017, -345.8246450283934905 ) ) ;
#52985=CARTESIAN_POINT ( 'NONE',  ( 17.69057799172644607, -295.8482004993076657, -319.5522096877774061 ) ) ;
#52986=CARTESIAN_POINT ( 'NONE',  ( -113.7950496592970779, -279.9615961741182559, -271.6169663873831155 ) ) ;
#52987=CARTESIAN_POINT ( 'NONE',  ( 35.50002531251338667, -291.8191611890306945, -289.6611138460939401 ) ) ;
#52988=CARTESIAN_POINT ( 'NONE',  ( -67.31108647503970133, -279.3147082179402219, -203.7597963752540124 ) ) ;
#52989=CARTESIAN_POINT ( 'NONE',  ( 34.46205805791058197, -293.3649064608505341, -242.4069416680160032 ) ) ;
#52990=CARTESIAN_POINT ( 'NONE',  ( -99.79227414052319034, -283.2047112595854514, -227.7335719275758663 ) ) ;
#52991=CARTESIAN_POINT ( 'NONE',  ( -98.01637611950918938, -279.9515046978928012, -314.4690477051376547 ) ) ;
#52992=CARTESIAN_POINT ( 'NONE',  ( -93.26982013910412661, -294.9409382661231689, -317.6611356547886089 ) ) ;
#52993=CARTESIAN_POINT ( 'NONE',  ( -30.68020254121020329, -296.1353836042920307, -195.3633804044103215 ) ) ;
#52996=CARTESIAN_POINT ( 'NONE',  ( 27.88413399525486369, -283.0466931843626526, -234.0645979971862118 ) ) ;
#52997=CARTESIAN_POINT ( 'NONE',  ( -109.3354294181779238, -296.2238419858752536, -257.9155812456735362 ) ) ;
#52999=CARTESIAN_POINT ( 'NONE',  ( -20.19161114001082069, -271.7666405000205714, -195.3683826091709363 ) ) ;
#53000=CARTESIAN_POINT ( 'NONE',  ( 1.123461091271782619, -273.7491908978996094, -203.8282707832596827 ) ) ;
#53001=CARTESIAN_POINT ( 'NONE',  ( 23.75853831036545927, -289.4843685441786647, -316.4052178972695515 ) ) ;
#53002=CARTESIAN_POINT ( 'NONE',  ( -107.3946968973942688, -290.6576443695460625, -249.7843809094832750 ) ) ;
#53003=CARTESIAN_POINT ( 'NONE',  ( -70.06543656954286803, -281.1331322640704684, -204.3178663081950504 ) ) ;
#53004=CARTESIAN_POINT ( 'NONE',  ( 96.68924888517000227, -301.5126242020289169, -196.3069997221729182 ) ) ;
#53005=CARTESIAN_POINT ( 'NONE',  ( -87.79248114618259535, -278.1233576937960379, -216.9818968792185956 ) ) ;
#53006=CARTESIAN_POINT ( 'NONE',  ( -102.7179183965434106, -272.9176807552647688, -229.6800402017144620 ) ) ;
#53007=CARTESIAN_POINT ( 'NONE',  ( -95.42965408058364574, -293.1176511800382514, -223.7886927239548527 ) ) ;
#53009=CARTESIAN_POINT ( 'NONE',  ( -108.2093379558849051, -291.4405548779228639, -252.3750077615254384 ) ) ;
#53011=CARTESIAN_POINT ( 'NONE',  ( -61.27555736024090294, -289.8843411434714312, -198.4207100790942491 ) ) ;
#53012=CARTESIAN_POINT ( 'NONE',  ( -90.05819054004119550, -296.9485288423666134, -219.7609553567533851 ) ) ;
#53014=CARTESIAN_POINT ( 'NONE',  ( -86.08515411122583316, -292.9109692148467161, -211.5831819810707941 ) ) ;
#53015=CARTESIAN_POINT ( 'NONE',  ( 40.65961533371913106, -290.2662352645559167, -288.1317622949166548 ) ) ;
#53016=CARTESIAN_POINT ( 'NONE',  ( 16.32701712819017459, -288.8167080040751102, -218.2104016491132938 ) ) ;
#53017=CARTESIAN_POINT ( 'NONE',  ( -0.5915648041198875440, -274.5628873244131114, -335.6075981082368003 ) ) ;
#53018=CARTESIAN_POINT ( 'NONE',  ( 34.29008848677463561, -277.7354209081919407, -290.6612418364263135 ) ) ;
#53019=CARTESIAN_POINT ( 'NONE',  ( -38.90375606591197055, -290.1122500275077414, -195.9375049135655615 ) ) ;
#53020=CARTESIAN_POINT ( 'NONE',  ( -79.24763684613134274, -281.3539909854462735, -207.1776680982772803 ) ) ;
#53022=CARTESIAN_POINT ( 'NONE',  ( -73.85489126903598844, -282.8990247954959614, -333.7487314242565617 ) ) ;
#53023=CARTESIAN_POINT ( 'NONE',  ( -114.0688391286936110, -279.6519961044837146, -268.7544982487737002 ) ) ;
#53024=CARTESIAN_POINT ( 'NONE',  ( -0.5795466856604392092, -281.3697773409666638, -337.5812819858398939 ) ) ;
#53025=CARTESIAN_POINT ( 'NONE',  ( -17.40741497080009026, -277.7422512970396156, -344.4923832326744559 ) ) ;
#53028=CARTESIAN_POINT ( 'NONE',  ( 11.32844739937061185, -276.2323756685872809, -211.5223723098345658 ) ) ;
#53029=CARTESIAN_POINT ( 'NONE',  ( 30.89617123739170168, -277.8376638359844719, -254.7536222014695397 ) ) ;
#53030=ORIENTED_EDGE ( 'NONE', *, *, #49884, .F. ) ;
#53032=CARTESIAN_POINT ( 'NONE',  ( -109.5208497428386494, -298.2901384315509858, -290.7368636486585842 ) ) ;
#53034=CARTESIAN_POINT ( 'NONE',  ( -8.082532586125303453, -289.7394651209468748, -337.6324074843216181 ) ) ;
#53035=CARTESIAN_POINT ( 'NONE',  ( -34.67957604879136824, -290.7792651970697761, -346.3011411006759772 ) ) ;
#53036=CARTESIAN_POINT ( 'NONE',  ( -36.19622276349792145, -291.4154381539049723, -197.2556659408412827 ) ) ;
#53037=CARTESIAN_POINT ( 'NONE',  ( 34.79870787013732070, -286.7214059749196622, -243.6162411466187621 ) ) ;
#53039=CARTESIAN_POINT ( 'NONE',  ( -96.57590147151967130, -282.3412929085624796, -314.3809976734893326 ) ) ;
#53040=CARTESIAN_POINT ( 'NONE',  ( -99.86962490730880404, -291.8682696704935893, -310.3751667958574672 ) ) ;
#53041=CARTESIAN_POINT ( 'NONE',  ( -108.6951794500373296, -283.2729355634384660, -251.9386115642138293 ) ) ;
#53043=CARTESIAN_POINT ( 'NONE',  ( -4.139662744114851023, -281.8145574705715717, -204.7813796066878922 ) ) ;
#53044=CARTESIAN_POINT ( 'NONE',  ( 7.805841084176246447, -289.3938539990620029, -332.5114538443609149 ) ) ;
#53045=CARTESIAN_POINT ( 'NONE',  ( -110.2204724192045973, -279.1125744993161106, -265.1965278867569964 ) ) ;
#53046=CARTESIAN_POINT ( 'NONE',  ( -74.47292207905763917, -290.3644405673160236, -203.3590204376128838 ) ) ;
#53047=CARTESIAN_POINT ( 'NONE',  ( -46.49642105660959857, -286.7415999113241583, -194.0699002380351885 ) ) ;
#53048=CARTESIAN_POINT ( 'NONE',  ( 2.703626289413516570, -287.0665495901047848, -204.6656178680383391 ) ) ;
#53049=CARTESIAN_POINT ( 'NONE',  ( -109.9946368399960903, -284.8192079691270351, -262.7521607666493537 ) ) ;
#53052=CARTESIAN_POINT ( 'NONE',  ( -22.45997228950932723, -294.1010007409788045, -196.0187729305145012 ) ) ;
#53053=CARTESIAN_POINT ( 'NONE',  ( 0.2832901835247852995, -293.2467705303265575, -336.9919503981581101 ) ) ;
#53054=CARTESIAN_POINT ( 'NONE',  ( -69.36509140515003935, -276.5428862207825773, -336.2378189899075664 ) ) ;
#53055=CARTESIAN_POINT ( 'NONE',  ( -112.4991034928404332, -296.1051980012548484, -254.0307771500460774 ) ) ;
#53056=CARTESIAN_POINT ( 'NONE',  ( 29.37436662899752804, -291.6117925792218557, -238.9408694813325553 ) ) ;
#53057=CARTESIAN_POINT ( 'NONE',  ( -109.7661201162576106, -294.9912530385681748, -255.0465033180652199 ) ) ;
#53058=CARTESIAN_POINT ( 'NONE',  ( -107.7806711441714782, -292.0291786409208612, -249.6892464931493407 ) ) ;
#53059=CARTESIAN_POINT ( 'NONE',  ( 8.431853164986209848, -295.4883968045187430, -327.6889906226460880 ) ) ;
#53061=CARTESIAN_POINT ( 'NONE',  ( -5.307539361340629647, -292.6314885058652067, -338.3740712721836417 ) ) ;
#53062=CARTESIAN_POINT ( 'NONE',  ( -11.08832550499942116, -300.3809508611794854, -195.3521588642121571 ) ) ;
#53063=CARTESIAN_POINT ( 'NONE',  ( 35.22763264693584517, -288.3589713167405648, -260.1371975069002929 ) ) ;
#53064=CARTESIAN_POINT ( 'NONE',  ( 34.50225496963312111, -277.8240175483897474, -293.0955174419003697 ) ) ;
#53065=CARTESIAN_POINT ( 'NONE',  ( 7.993650690917188051, -275.2431296414775943, -332.1739661845221008 ) ) ;
#53066=CARTESIAN_POINT ( 'NONE',  ( -2.596169063361186247, -273.8480426571001658, -201.7456988806351887 ) ) ;
#53067=CARTESIAN_POINT ( 'NONE',  ( 37.00287235400327290, -279.6807381723089634, -274.1292392309097181 ) ) ;
#53068=CARTESIAN_POINT ( 'NONE',  ( -35.74887623184653052, -275.4323944858504092, -346.5574588081581169 ) ) ;
#53069=CARTESIAN_POINT ( 'NONE',  ( -110.5398752692821063, -295.3303424341170285, -263.2352950540829966 ) ) ;
#53070=CARTESIAN_POINT ( 'NONE',  ( -106.3221749556402642, -274.9386761118286699, -240.7908190081843713 ) ) ;
#53071=CARTESIAN_POINT ( 'NONE',  ( -93.86247401662384959, -273.8595552451971002, -223.9810552638743957 ) ) ;
#53073=CARTESIAN_POINT ( 'NONE',  ( -111.7402384325737330, -288.4193012115740657, -282.3304246411586291 ) ) ;
#53074=CARTESIAN_POINT ( 'NONE',  ( -43.48000795694964893, -273.8059169533816544, -197.5689391568368194 ) ) ;
#53075=CARTESIAN_POINT ( 'NONE',  ( 39.35466548195799419, -287.4595567307200668, -262.9572619183762185 ) ) ;
#53076=CARTESIAN_POINT ( 'NONE',  ( -26.53034998962469970, -300.1667386724928974, -195.0022827325802837 ) ) ;
#53077=CARTESIAN_POINT ( 'NONE',  ( -74.22770907569548626, -293.5435474187963223, -335.4721828747001382 ) ) ;
#53078=CARTESIAN_POINT ( 'NONE',  ( -97.92343253587729635, -283.1164804569623925, -317.6264596162449152 ) ) ;
#53080=CARTESIAN_POINT ( 'NONE',  ( 24.49356269736469116, -280.1281015268789361, -312.8931178943216764 ) ) ;
#53082=CARTESIAN_POINT ( 'NONE',  ( -99.18454879530479218, -288.8032722392601954, -309.8907596876761090 ) ) ;
#53083=CARTESIAN_POINT ( 'NONE',  ( -94.38618975279069900, -282.0289136621867669, -317.8668196045017567 ) ) ;
#53085=CARTESIAN_POINT ( 'NONE',  ( -111.3978944739675967, -288.3986596511339258, -282.3029557302596686 ) ) ;
#53086=CARTESIAN_POINT ( 'NONE',  ( -64.84535885508721265, -275.2064405000169813, -201.9789738510249606 ) ) ;
#53087=CARTESIAN_POINT ( 'NONE',  ( -94.09460407729157794, -285.0544610868515178, -321.8307052268637563 ) ) ;
#53088=CARTESIAN_POINT ( 'NONE',  ( -68.23255946046616316, -271.7294917379506956, -201.3899860719557182 ) ) ;
#53089=CARTESIAN_POINT ( 'NONE',  ( -108.0932257389820847, -284.3148596790021543, -288.3394834179954955 ) ) ;
#53090=CARTESIAN_POINT ( 'NONE',  ( 5.756450122681592951, -277.8808192620658133, -330.0723936471982825 ) ) ;
#53091=CARTESIAN_POINT ( 'NONE',  ( 31.41702368083613450, -276.6890631944721122, -295.5051851116778039 ) ) ;
#53092=CARTESIAN_POINT ( 'NONE',  ( 20.98441271096739413, -284.2015567171311545, -317.5307825527482919 ) ) ;
#53094=CARTESIAN_POINT ( 'NONE',  ( -111.3722443963805944, -270.7948086242133741, -270.3387427897214366 ) ) ;
#53095=CARTESIAN_POINT ( 'NONE',  ( -19.28934018835978037, -294.6595437023015620, -345.2699430561930285 ) ) ;
#53097=CARTESIAN_POINT ( 'NONE',  ( 36.90796428035401533, -289.4330935638645315, -262.6907766247290397 ) ) ;
#53099=CARTESIAN_POINT ( 'NONE',  ( 25.22466315766302358, -290.4094976428775112, -220.5068182859052968 ) ) ;
#53100=CARTESIAN_POINT ( 'NONE',  ( -99.17047664396717721, -278.0777680996212098, -224.9661163902325995 ) ) ;
#53101=CARTESIAN_POINT ( 'NONE',  ( -25.12936684835842627, -290.6052608892674129, -195.1460973443744535 ) ) ;
#53103=CARTESIAN_POINT ( 'NONE',  ( -106.2197743360474789, -286.4188098488127139, -244.1596171725175282 ) ) ;
#53104=CARTESIAN_POINT ( 'NONE',  ( -104.2959747123585714, -280.7341000127553912, -238.6953854289459684 ) ) ;
#53105=CARTESIAN_POINT ( 'NONE',  ( -5.039664744714470679, -287.8943973664414102, -201.1138450738742165 ) ) ;
#53106=CARTESIAN_POINT ( 'NONE',  ( 25.82836802917675101, -284.0977715741896077, -310.8861224016510505 ) ) ;
#53107=CARTESIAN_POINT ( 'NONE',  ( 38.73609110630037122, -275.8716117948317219, -282.5773027869169027 ) ) ;
#53108=CARTESIAN_POINT ( 'NONE',  ( -61.01415464943616485, -295.7636101426791129, -199.5147726885362829 ) ) ;
#53109=CARTESIAN_POINT ( 'NONE',  ( -112.7171070979885172, -278.5830350032547358, -254.5638826296090542 ) ) ;
#53110=CARTESIAN_POINT ( 'NONE',  ( -39.22887118328734601, -299.9484728844831238, -195.9323858445324618 ) ) ;
#53112=CARTESIAN_POINT ( 'NONE',  ( 35.77081079830085031, -277.8376638359845288, -253.6410175316879361 ) ) ;
#53113=CARTESIAN_POINT ( 'NONE',  ( -79.91111264041815332, -295.6230357541203375, -207.6230913565478318 ) ) ;
#53114=CARTESIAN_POINT ( 'NONE',  ( 202.9738562182569694, 291.9636489450776367, -53.99999999998589573 ) ) ;
#53115=CARTESIAN_POINT ( 'NONE',  ( -78.67197487995659344, -277.1329472997456378, -330.6705213806835104 ) ) ;
#53116=CARTESIAN_POINT ( 'NONE',  ( -58.02921237668380172, -274.9958717929322347, -196.5493790434523476 ) ) ;
#53117=CARTESIAN_POINT ( 'NONE',  ( 38.43364710046513721, -280.7660423054147145, -282.7279770925704270 ) ) ;
#53118=CARTESIAN_POINT ( 'NONE',  ( -69.17376816947050600, -291.2369097079285893, -337.1794796870520372 ) ) ;
#53119=CARTESIAN_POINT ( 'NONE',  ( -107.7279442483919780, -297.6924742345010486, -299.9678498616898423 ) ) ;
#53120=CARTESIAN_POINT ( 'NONE',  ( -113.3824888224443157, -297.8736747972851049, -261.0979018603624695 ) ) ;
#53121=CARTESIAN_POINT ( 'NONE',  ( 20.75333946067408775, -294.9010370192700634, -223.1710098276439282 ) ) ;
#53122=CARTESIAN_POINT ( 'NONE',  ( 20.75973241486496690, -280.2031966318053264, -317.5432843601915351 ) ) ;
#53123=CARTESIAN_POINT ( 'NONE',  ( 34.49695675517361337, -283.2190327955023008, -250.8054480651313440 ) ) ;
#53124=CARTESIAN_POINT ( 'NONE',  ( -111.2067164228949849, -270.7156358070457713, -259.2473669982903743 ) ) ;
#53125=CARTESIAN_POINT ( 'NONE',  ( -112.2160862844201716, -286.3345478224298404, -255.9346161509436968 ) ) ;
#53126=CARTESIAN_POINT ( 'NONE',  ( 35.58328662822450639, -286.3740230092009824, -262.8662944469925264 ) ) ;
#53127=CARTESIAN_POINT ( 'NONE',  ( 7.222567447766102156, -59.30128903974464549, -354.3697514511841291 ) ) ;
#53129=CARTESIAN_POINT ( 'NONE',  ( 28.38757444900029014, -286.6384726524639177, -309.3260862918506859 ) ) ;
#53130=CARTESIAN_POINT ( 'NONE',  ( 30.99588644589087139, -286.8739020207829640, -244.4877991421641354 ) ) ;
#53132=CARTESIAN_POINT ( 'NONE',  ( -8.143784945859268376, -283.7583993691098385, -341.3326965424229797 ) ) ;
#53133=CARTESIAN_POINT ( 'NONE',  ( 32.87917625717777526, -275.6185522417418383, -250.1525995261814046 ) ) ;
#53134=CARTESIAN_POINT ( 'NONE',  ( -25.05735290322474640, -291.1256340710792756, -194.6604751697547329 ) ) ;
#53135=CARTESIAN_POINT ( 'NONE',  ( 33.47530174809608638, -282.5870429639839472, -300.4682081209094804 ) ) ;
#53137=CARTESIAN_POINT ( 'NONE',  ( 37.30236197100010287, -282.8715525308364249, -254.4565934074510380 ) ) ;
#53138=CARTESIAN_POINT ( 'NONE',  ( 24.24074137218694958, -282.5003303425487502, -316.5492895254176346 ) ) ;
#53139=CARTESIAN_POINT ( 'NONE',  ( -5.558494192811491708, -280.4822903412832602, -204.6433287586655183 ) ) ;
#53140=CARTESIAN_POINT ( 'NONE',  ( 27.33386217378598815, -291.4809262143062369, -301.5434626090942629 ) ) ;
#53141=CARTESIAN_POINT ( 'NONE',  ( 139.4746202765078635, 180.3694368708648881, -241.5727912977973517 ) ) ;
#53142=ORIENTED_EDGE ( 'NONE', *, *, #20462, .F. ) ;
#53143=CARTESIAN_POINT ( 'NONE',  ( 12.99937841255446891, -278.3477951860328972, -325.8011604366477627 ) ) ;
#53144=CARTESIAN_POINT ( 'NONE',  ( 184.6061638061233623, 263.7319966466967571, -153.1343895057649149 ) ) ;
#53145=CARTESIAN_POINT ( 'NONE',  ( 18.30545796200765452, -278.8762099623819495, -220.6093280588681296 ) ) ;
#53146=CARTESIAN_POINT ( 'NONE',  ( -66.85289343556999597, -297.0035275889329682, -203.4670629724890887 ) ) ;
#53147=CARTESIAN_POINT ( 'NONE',  ( 4.113661539522734500, -292.1020349893318553, -205.4829984225391968 ) ) ;
#53148=CARTESIAN_POINT ( 'NONE',  ( 6.586641810477393832, -59.71310429701481581, -351.1713004201100716 ) ) ;
#53149=CARTESIAN_POINT ( 'NONE',  ( -113.6876631197567207, -271.3089124547065012, -264.6462902796607750 ) ) ;
#53150=CARTESIAN_POINT ( 'NONE',  ( -111.1675578940935480, -288.9773369555932732, -268.4206126772065204 ) ) ;
#53151=CARTESIAN_POINT ( 'NONE',  ( -94.88522819567236866, -297.7594964438854390, -317.2810664774769407 ) ) ;
#53152=CARTESIAN_POINT ( 'NONE',  ( 0.4076873518200785917, -287.8812678645984420, -207.2444627014909315 ) ) ;
#53154=CARTESIAN_POINT ( 'NONE',  ( 8.700195859958466116, -293.6068816611182228, -208.8703248258991607 ) ) ;
#53155=CARTESIAN_POINT ( 'NONE',  ( -97.41010596873425698, -285.6237138482405840, -228.7484364484415380 ) ) ;
#53156=CARTESIAN_POINT ( 'NONE',  ( -87.19216369623259766, -296.1706932979686258, -212.1281569087043692 ) ) ;
#53157=CARTESIAN_POINT ( 'NONE',  ( -30.72139348939228043, -292.9365220751944889, -193.7556757403533823 ) ) ;
#53158=CARTESIAN_POINT ( 'NONE',  ( -7.220078199748824588, -292.9291235076543671, -199.5498112497721479 ) ) ;
#53159=CARTESIAN_POINT ( 'NONE',  ( -108.9383144368351282, -290.5300720249093729, -284.6702148773316594 ) ) ;
#53162=CARTESIAN_POINT ( 'NONE',  ( -65.11169700461144316, -299.5536969880821516, -199.8129591888135792 ) ) ;
#53163=CARTESIAN_POINT ( 'NONE',  ( -93.84197009086221897, -272.0544989609218192, -218.6143137164453378 ) ) ;
#53165=CARTESIAN_POINT ( 'NONE',  ( 21.19075931006214120, -281.2272264910766921, -314.3972846656168940 ) ) ;
#53167=VERTEX_POINT ( 'NONE', #69083 ) ;
#53168=CARTESIAN_POINT ( 'NONE',  ( -20.14596317591239583, -276.3447053597206491, -345.4080151431380159 ) ) ;
#53169=CARTESIAN_POINT ( 'NONE',  ( -110.9855806072527145, -271.0241451809015985, -264.8334572699994851 ) ) ;
#53170=CARTESIAN_POINT ( 'NONE',  ( -101.8974378896173363, -280.9061790864847694, -233.7083936606909162 ) ) ;
#53171=CARTESIAN_POINT ( 'NONE',  ( 20.12295111955519644, -274.3463404851326004, -317.3777291786734054 ) ) ;
#53173=CARTESIAN_POINT ( 'NONE',  ( -110.4936033283150749, -297.6707798004966889, -276.9504786201209754 ) ) ;
#53174=CARTESIAN_POINT ( 'NONE',  ( -110.5769942451401704, -273.4932526910073989, -270.3730743911539776 ) ) ;
#53175=CARTESIAN_POINT ( 'NONE',  ( -54.43572055365810769, -299.4362059628888915, -196.1032235936009727 ) ) ;
#53176=CARTESIAN_POINT ( 'NONE',  ( 16.92304405480740215, -272.8400972220205745, -218.0009651343474957 ) ) ;
#53177=CARTESIAN_POINT ( 'NONE',  ( -4.283151202243660194, -295.2558588116890519, -335.5750214408553234 ) ) ;
#53178=CARTESIAN_POINT ( 'NONE',  ( -38.89194050737955166, -290.6070517462883345, -196.7882175810221952 ) ) ;
#53180=CARTESIAN_POINT ( 'NONE',  ( -51.29529987717894102, -277.7183217067786245, -346.0236844015495308 ) ) ;
#53181=CARTESIAN_POINT ( 'NONE',  ( -39.17311196632604009, -298.3618566532203999, -197.3505314855477479 ) ) ;
#53183=CARTESIAN_POINT ( 'NONE',  ( 4.263380231796848108, -281.1890568535980606, -334.6289856000636860 ) ) ;
#53184=CARTESIAN_POINT ( 'NONE',  ( 23.41969440745005571, -296.1541468766243383, -314.6330216019263162 ) ) ;
#53187=CARTESIAN_POINT ( 'NONE',  ( -65.38703105931877246, -282.6255385255211081, -337.9473835880162369 ) ) ;
#53188=CARTESIAN_POINT ( 'NONE',  ( -111.7873673732580357, -282.4142092780639928, -281.1157403056614044 ) ) ;
#53189=CARTESIAN_POINT ( 'NONE',  ( 27.16168139506032730, -273.6456624114957776, -234.8332814406924740 ) ) ;
#53190=CARTESIAN_POINT ( 'NONE',  ( 23.91032801655921958, -282.9640423458236569, -227.0588760057046613 ) ) ;
#53193=CARTESIAN_POINT ( 'NONE',  ( -21.50100266378104052, -272.6518762875633115, -195.8258061011742086 ) ) ;
#53194=CARTESIAN_POINT ( 'NONE',  ( -79.18398686719039858, -279.6149906439246138, -332.8677480620823417 ) ) ;
#53195=DIRECTION ( 'NONE',  ( -1.000000000000000000, -0.000000000000000000, -0.000000000000000000 ) ) ;
#53196=CARTESIAN_POINT ( 'NONE',  ( -70.45759954843084927, -287.5391475790112850, -202.4446147732228951 ) ) ;
#53198=CARTESIAN_POINT ( 'NONE',  ( -111.7067687828262166, -288.6819412171976182, -260.2402206439201109 ) ) ;
#53200=CARTESIAN_POINT ( 'NONE',  ( -108.5564991955320266, -295.5808450781406123, -252.5450553201070250 ) ) ;
#53201=CARTESIAN_POINT ( 'NONE',  ( -76.54074725841762472, -287.7222619714048051, -333.4031688978202510 ) ) ;
#53202=CARTESIAN_POINT ( 'NONE',  ( -72.76141013609318975, -193.8959084914727669, -354.0272458012134393 ) ) ;
#53203=CARTESIAN_POINT ( 'NONE',  ( -111.3402603691592674, -294.3951485864391771, -282.5764252751562253 ) ) ;
#53204=CARTESIAN_POINT ( 'NONE',  ( 38.10302698336676741, -285.8866013197556981, -258.8371542206519962 ) ) ;
#53205=CARTESIAN_POINT ( 'NONE',  ( 28.48585653638552984, -282.7028302378168974, -236.8836160027974245 ) ) ;
#53206=CARTESIAN_POINT ( 'NONE',  ( -47.14808262679986939, -281.4149660246019380, -345.7123546981116533 ) ) ;
#53207=CARTESIAN_POINT ( 'NONE',  ( -94.29090639493006165, -291.1978081416179407, -224.6708273778320972 ) ) ;
#53208=CARTESIAN_POINT ( 'NONE',  ( 31.61614055084014652, -282.6357301102995052, -244.5208381995067271 ) ) ;
#53209=CARTESIAN_POINT ( 'NONE',  ( 35.59088192707488219, -282.4391504593885429, -276.7551007935517191 ) ) ;
#53210=CARTESIAN_POINT ( 'NONE',  ( 17.46619677065141119, -290.2536437759505930, -322.0766982301693133 ) ) ;
#53211=CARTESIAN_POINT ( 'NONE',  ( -97.79909679341338347, -273.5229275846163546, -222.7098065618112059 ) ) ;
#53212=CARTESIAN_POINT ( 'NONE',  ( 18.54243952888901958, -286.3365617539775485, -321.2358361579501889 ) ) ;
#53213=CARTESIAN_POINT ( 'NONE',  ( 31.25029666173524845, -275.1015462326435568, -235.3734347728104694 ) ) ;
#53214=CARTESIAN_POINT ( 'NONE',  ( 28.93565103743292966, -295.0753337591519880, -236.0222257148051597 ) ) ;
#53216=CARTESIAN_POINT ( 'NONE',  ( 10.59707575819634329, -283.1948066931273047, -210.1954327657594490 ) ) ;
#53217=CARTESIAN_POINT ( 'NONE',  ( 30.19655231208273705, -273.9873451788620287, -303.4737239230440196 ) ) ;
#53219=CARTESIAN_POINT ( 'NONE',  ( -104.5384193880964006, -295.4225277694550300, -234.3181771353212355 ) ) ;
#53220=CARTESIAN_POINT ( 'NONE',  ( -110.0686411521480608, -292.3197179683884315, -257.5296459578963209 ) ) ;
#53221=CARTESIAN_POINT ( 'NONE',  ( -74.31779062108446965, -272.8954765581785296, -207.2417080407740286 ) ) ;
#53222=CARTESIAN_POINT ( 'NONE',  ( -92.20213089438688314, -292.7699762491427009, -221.1381636908673158 ) ) ;
#53223=CARTESIAN_POINT ( 'NONE',  ( -86.09457117559314554, -292.2979480365151517, -215.6433673060070930 ) ) ;
#53224=CARTESIAN_POINT ( 'NONE',  ( -110.6185932857513166, -286.4478074503168727, -259.9461795396508705 ) ) ;
#53225=CARTESIAN_POINT ( 'NONE',  ( -111.0690885312376821, -292.2313127495139611, -250.2395914609065812 ) ) ;
#53226=CARTESIAN_POINT ( 'NONE',  ( -27.92649790953471367, -293.4843411741887849, -194.3824814416859681 ) ) ;
#53227=CARTESIAN_POINT ( 'NONE',  ( 14.31477911683075988, -294.1346789447569563, -322.0132735675327922 ) ) ;
#53228=CARTESIAN_POINT ( 'NONE',  ( 35.97096331013060677, -289.7561556857563119, -286.2408678831799307 ) ) ;
#53229=CARTESIAN_POINT ( 'NONE',  ( 36.17507721616056671, -281.4311824980786696, -247.4638811749261436 ) ) ;
#53230=CARTESIAN_POINT ( 'NONE',  ( -103.1447997570861190, -271.1886675844338015, -232.7024905364028768 ) ) ;
#53231=CARTESIAN_POINT ( 'NONE',  ( -112.2196487879977838, -284.1602541102888040, -288.3694544525799870 ) ) ;
#53232=CARTESIAN_POINT ( 'NONE',  ( 34.83900185257586912, -277.7776690860425788, -289.3819767158265677 ) ) ;
#53234=CARTESIAN_POINT ( 'NONE',  ( -102.1289017722122310, -282.8782940458734174, -304.9620689189410996 ) ) ;
#53235=CARTESIAN_POINT ( 'NONE',  ( 19.94447813150229365, -286.2215906952047249, -318.7687044986275282 ) ) ;
#53236=CARTESIAN_POINT ( 'NONE',  ( -95.22116186246697112, -276.0221612431938638, -319.2715726048051010 ) ) ;
#53237=CARTESIAN_POINT ( 'NONE',  ( 144.2857639756989272, -299.5541904835127980, -195.3611179825600175 ) ) ;
#53239=CARTESIAN_POINT ( 'NONE',  ( -88.94218930997929817, -283.3087520617530117, -322.1561914821513142 ) ) ;
#53240=STYLED_ITEM('',(#93745),#58557);
#53241=CARTESIAN_POINT ( 'NONE',  ( -94.67484783465863529, -280.4490567075629315, -219.5583730451570830 ) ) ;
#53242=CARTESIAN_POINT ( 'NONE',  ( 27.24033664975637237, -287.1580777940153553, -311.9558621771410571 ) ) ;
#53243=CARTESIAN_POINT ( 'NONE',  ( 35.84337314420839959, -295.4603078293741305, -281.7368349655928341 ) ) ;
#53244=CARTESIAN_POINT ( 'NONE',  ( 23.82539689038724617, -276.5416842638102821, -224.9185535801931621 ) ) ;
#53245=CARTESIAN_POINT ( 'NONE',  ( 36.41469916907177407, -277.1241894832037929, -290.7395866213784075 ) ) ;
#53246=CARTESIAN_POINT ( 'NONE',  ( -27.02361157036015626, -276.7506197147289413, -342.6282408878328170 ) ) ;
#53247=CARTESIAN_POINT ( 'NONE',  ( -95.91880397987304718, -275.1704977573533029, -224.0948266738041923 ) ) ;
#53248=CARTESIAN_POINT ( 'NONE',  ( 34.02960341810776868, -285.2605713031388746, -247.8200497228821177 ) ) ;
#53249=AXIS2_PLACEMENT_3D ( 'NONE', #48314, #5725, #34600 ) ;
#53250=CARTESIAN_POINT ( 'NONE',  ( -92.99443189435838519, -291.4342873639084814, -322.4872485198813479 ) ) ;
#53251=CARTESIAN_POINT ( 'NONE',  ( -7.876631510554272353, -293.5770968422284000, -337.5017639540419054 ) ) ;
#53253=CARTESIAN_POINT ( 'NONE',  ( -69.02293574344011517, -291.2904329886188179, -204.5568346340573100 ) ) ;
#53255=CARTESIAN_POINT ( 'NONE',  ( -87.17310460768425173, -290.8069482824485590, -328.7260013536424594 ) ) ;
#53256=CARTESIAN_POINT ( 'NONE',  ( -108.3906952617237778, -279.4302199975909389, -253.1584158969775729 ) ) ;
#53257=CARTESIAN_POINT ( 'NONE',  ( -112.9017446749930542, -295.3039497443256778, -283.7829506566654345 ) ) ;
#53258=CARTESIAN_POINT ( 'NONE',  ( 37.92202597641377793, -288.0052802938665764, -254.5276652446351591 ) ) ;
#53260=CARTESIAN_POINT ( 'NONE',  ( 37.12503845127565683, -288.1296532977685274, -289.8662233899973444 ) ) ;
#53261=CARTESIAN_POINT ( 'NONE',  ( -108.0501975829110535, -285.1260389607461434, -252.1293908419040122 ) ) ;
#53262=CARTESIAN_POINT ( 'NONE',  ( 84.36106466651209246, 83.41242399426737109, -302.2512376199425717 ) ) ;
#53263=CARTESIAN_POINT ( 'NONE',  ( 195.6868322499005046, 284.9009392118488790, -111.2773971726515470 ) ) ;
#53264=CARTESIAN_POINT ( 'NONE',  ( -108.1557645722374303, -264.0394726077588530, -305.3744954675115650 ) ) ;
#53265=CARTESIAN_POINT ( 'NONE',  ( -92.85582339289652509, -277.0723915473839156, -318.0138602488598849 ) ) ;
#53266=CARTESIAN_POINT ( 'NONE',  ( -110.4777982728515013, -277.3972277977297836, -276.0894038606994059 ) ) ;
#53267=CARTESIAN_POINT ( 'NONE',  ( -101.1886334701071064, -272.7866564770629338, -227.2625840664813666 ) ) ;
#53268=CARTESIAN_POINT ( 'NONE',  ( -101.2118702128279324, -255.6233436704357018, -324.8885547363302067 ) ) ;
#53269=CARTESIAN_POINT ( 'NONE',  ( -9.407574802891977228, -275.3793965981718088, -341.5859936591876931 ) ) ;
#53270=CARTESIAN_POINT ( 'NONE',  ( -104.1013986831535334, -290.6437312344595512, -300.1698877893368262 ) ) ;
#53271=CARTESIAN_POINT ( 'NONE',  ( 76.08029918769435085, -300.2411797159293769, -193.5075115251480895 ) ) ;
#53272=CARTESIAN_POINT ( 'NONE',  ( 36.14815395606711945, -286.2460945185633818, -271.0574104906677917 ) ) ;
#53273=CARTESIAN_POINT ( 'NONE',  ( -3.450481238932981753, -298.9581682151539894, -193.4199041260204410 ) ) ;
#53274=CARTESIAN_POINT ( 'NONE',  ( -90.40577614855953925, -295.9960482218384072, -320.5657778681049308 ) ) ;
#53276=CARTESIAN_POINT ( 'NONE',  ( -59.22417564993066463, -279.2533840340722691, -342.6831164397335101 ) ) ;
#53278=CARTESIAN_POINT ( 'NONE',  ( 38.36389194211682963, -281.2324255043786252, -284.1525077467491087 ) ) ;
#53280=CARTESIAN_POINT ( 'NONE',  ( -96.66389756162209324, -280.2320419986169782, -227.2902117246974285 ) ) ;
#53281=CARTESIAN_POINT ( 'NONE',  ( -62.05495501160649496, -279.1291277436454834, -342.2722915213602164 ) ) ;
#53282=CARTESIAN_POINT ( 'NONE',  ( -90.45870103370764070, -295.8567138240070449, -219.3572883281996724 ) ) ;
#53284=CARTESIAN_POINT ( 'NONE',  ( -96.09174159185934627, -278.1112956120808803, -313.7114205486456626 ) ) ;
#53285=CARTESIAN_POINT ( 'NONE',  ( -105.4705123126592667, -273.8156153054890183, -234.7126731335976899 ) ) ;
#53286=CARTESIAN_POINT ( 'NONE',  ( 16.63212666722990463, -276.8195081145228755, -218.2113917777019765 ) ) ;
#53287=CARTESIAN_POINT ( 'NONE',  ( 25.57133689010938937, -274.7048791307898341, -313.8180464572321853 ) ) ;
#53289=CARTESIAN_POINT ( 'NONE',  ( -102.9948276916164076, -289.3128295293842029, -302.6453024626476918 ) ) ;
#53291=CARTESIAN_POINT ( 'NONE',  ( -97.49547028825384132, -284.5429643603194449, -222.4566638813180646 ) ) ;
#53292=CARTESIAN_POINT ( 'NONE',  ( 22.95182841329831902, -279.2006047116560694, -227.4348506080987420 ) ) ;
#53293=CARTESIAN_POINT ( 'NONE',  ( 34.51184905986551854, -280.3347945101170353, -286.2495536558953404 ) ) ;
#53294=CARTESIAN_POINT ( 'NONE',  ( -40.00135534845858842, -284.0983164198792679, -195.9686423258791024 ) ) ;
#53295=CARTESIAN_POINT ( 'NONE',  ( -8.371534899360042914, -290.6730724307741411, -339.5537669755875072 ) ) ;
#53296=CARTESIAN_POINT ( 'NONE',  ( -46.52125161606375059, -281.1382826988426586, -197.4889545147629804 ) ) ;
#53297=CARTESIAN_POINT ( 'NONE',  ( -95.79649060784740300, -239.9130894949069273, -341.7038789641651420 ) ) ;
#53299=CARTESIAN_POINT ( 'NONE',  ( -73.91016683735213633, -281.9289795067448381, -337.2719819784207402 ) ) ;
#53300=CARTESIAN_POINT ( 'NONE',  ( 36.63783524064525920, -295.7116295160258232, -282.7690944289590220 ) ) ;
#53301=CARTESIAN_POINT ( 'NONE',  ( -86.13662427978462688, -277.6264869320473281, -212.0428378762436239 ) ) ;
#53302=CARTESIAN_POINT ( 'NONE',  ( -60.63866816184651043, -285.3536961940569654, -341.8807036344308017 ) ) ;
#53305=CARTESIAN_POINT ( 'NONE',  ( -28.05086643719268835, -294.0892237539399048, -195.3218194102945517 ) ) ;
#53307=CARTESIAN_POINT ( 'NONE',  ( 35.45645305944830028, -273.3202936041259363, -252.3214521044563980 ) ) ;
#53308=CARTESIAN_POINT ( 'NONE',  ( 37.34504015396549192, -286.9762866145327962, -288.4735153254003990 ) ) ;
#53309=CARTESIAN_POINT ( 'NONE',  ( -105.4334054509244538, -289.3312277487780761, -241.7684228450832506 ) ) ;
#53311=CARTESIAN_POINT ( 'NONE',  ( 35.59335598344972595, -274.3607329713705099, -279.8062133709154864 ) ) ;
#53312=CARTESIAN_POINT ( 'NONE',  ( -20.59213019760519714, -292.9745255301173756, -342.7350333072060380 ) ) ;
#53313=CARTESIAN_POINT ( 'NONE',  ( -108.5906737121535457, -292.1042083185274691, -252.2869241974576937 ) ) ;
#53316=CARTESIAN_POINT ( 'NONE',  ( 38.91330782135023014, -292.0674607705779522, -273.1685213399239274 ) ) ;
#53317=CARTESIAN_POINT ( 'NONE',  ( 35.31282047177651151, -289.3212938334405635, -283.3133785098077624 ) ) ;
#53318=CARTESIAN_POINT ( 'NONE',  ( 2.627798813909436149, -286.7642557421354468, -335.0480066675617081 ) ) ;
#53319=CARTESIAN_POINT ( 'NONE',  ( 34.27962083901346091, -288.7555012119815387, -253.4022385556386041 ) ) ;
#53321=CARTESIAN_POINT ( 'NONE',  ( 25.08318942048913769, -287.8304560759564197, -232.2070239481237195 ) ) ;
#53322=CARTESIAN_POINT ( 'NONE',  ( 12.33096567822983936, -296.3449497253816389, -327.0963018696066342 ) ) ;
#53324=CARTESIAN_POINT ( 'NONE',  ( -29.51882367111351257, -287.3542226296139575, -194.1586815245778723 ) ) ;
#53325=CARTESIAN_POINT ( 'NONE',  ( -45.51855283331879320, -275.2347078105296418, -345.5294498129835006 ) ) ;
#53326=CARTESIAN_POINT ( 'NONE',  ( -112.1536246696261827, -278.6578606600517674, -288.5524745620706426 ) ) ;
#53327=CARTESIAN_POINT ( 'NONE',  ( -45.26697170667152648, -279.6212228549536576, -193.7383416711709572 ) ) ;
#53328=CARTESIAN_POINT ( 'NONE',  ( -109.7770570454589460, -298.7652977454988559, -252.2819061632672799 ) ) ;
#53329=CARTESIAN_POINT ( 'NONE',  ( -42.79480560662226196, -283.9831991590132247, -195.5466472428230134 ) ) ;
#53331=CARTESIAN_POINT ( 'NONE',  ( -71.48911177423597962, -277.7357922077416106, -204.4315472810838799 ) ) ;
#53332=CARTESIAN_POINT ( 'NONE',  ( -87.01645424888360481, -281.7431171264859131, -326.6214025603719051 ) ) ;
#53334=CARTESIAN_POINT ( 'NONE',  ( 22.08871162433874957, -274.6795556270596990, -318.2433910655992122 ) ) ;
#53335=CARTESIAN_POINT ( 'NONE',  ( -104.3570865205281422, -298.4832359403894770, -239.5845805086292444 ) ) ;
#53337=CARTESIAN_POINT ( 'NONE',  ( -41.56591789986394758, -282.0243770713628351, -346.9876977603199180 ) ) ;
#53338=CARTESIAN_POINT ( 'NONE',  ( -96.29684121857637535, -298.1006036656422111, -226.8922746056790061 ) ) ;
#53339=CARTESIAN_POINT ( 'NONE',  ( -37.27096458327439166, -299.3681896575296264, -193.8534906611272675 ) ) ;
#53340=CARTESIAN_POINT ( 'NONE',  ( -48.87459184230568354, -273.5680489240326665, -198.2052845423936276 ) ) ;
#53341=CARTESIAN_POINT ( 'NONE',  ( 24.98963354731172259, -294.9884647040649384, -228.6501423155503403 ) ) ;
#53342=CARTESIAN_POINT ( 'NONE',  ( 31.68836297362905086, -288.1585853358938039, -304.5966267694757335 ) ) ;
#53343=CARTESIAN_POINT ( 'NONE',  ( -25.59488731868887612, -278.2805586575643133, -195.7197984296246318 ) ) ;
#53344=CARTESIAN_POINT ( 'NONE',  ( -100.0298143814077889, -290.9776920624801733, -225.6486998431002746 ) ) ;
#53346=CARTESIAN_POINT ( 'NONE',  ( -3.267544394144144437, -287.6496402726385213, -335.2428918257706982 ) ) ;
#53347=CARTESIAN_POINT ( 'NONE',  ( 35.15604847583838932, -291.3044901863527798, -251.1001245313546519 ) ) ;
#53348=ORIENTED_EDGE ( 'NONE', *, *, #20584, .T. ) ;
#53349=FACE_OUTER_BOUND ( 'NONE', #80054, .T. ) ;
#53350=CARTESIAN_POINT ( 'NONE',  ( 35.02045035014045027, -287.1939285195435900, -280.5371703710089264 ) ) ;
#53352=CARTESIAN_POINT ( 'NONE',  ( -95.64572995639733222, -286.1699047810917023, -220.3468183581427695 ) ) ;
#53353=CARTESIAN_POINT ( 'NONE',  ( 37.83393706612440610, -292.4151704371259370, -254.7581827960663361 ) ) ;
#53354=CARTESIAN_POINT ( 'NONE',  ( -22.67721911498254528, -281.5511009678966161, -195.2189220750527738 ) ) ;
#53355=CARTESIAN_POINT ( 'NONE',  ( -26.74487334013010553, -282.7470670097438301, -342.6391941126705660 ) ) ;
#53356=CARTESIAN_POINT ( 'NONE',  ( -62.84504740938675837, -297.7290993848732228, -197.7072861672377257 ) ) ;
#53357=CARTESIAN_POINT ( 'NONE',  ( -62.21222647214859336, -275.0369775354597550, -201.2040475043935146 ) ) ;
#53358=CARTESIAN_POINT ( 'NONE',  ( -25.11539492085915981, -290.2287740458283452, -196.6717721318000827 ) ) ;
#53359=CARTESIAN_POINT ( 'NONE',  ( -64.70263319476210029, -272.4816827481196810, -202.2409597299379413 ) ) ;
#53362=CARTESIAN_POINT ( 'NONE',  ( -40.05032774112678595, -287.9380037307938096, -195.9704093108784662 ) ) ;
#53364=CARTESIAN_POINT ( 'NONE',  ( -58.75178810823440045, -296.4022886058531867, -344.0581684737222758 ) ) ;
#53365=CARTESIAN_POINT ( 'NONE',  ( -109.5978189156831348, -285.0532267569257101, -281.7737427951699374 ) ) ;
#53366=CARTESIAN_POINT ( 'NONE',  ( 39.14504054577020753, -274.6927786480415534, -276.8878869815503663 ) ) ;
#53367=CARTESIAN_POINT ( 'NONE',  ( 38.25857087792454081, -294.3806283060176838, -284.5004208082049217 ) ) ;
#53368=CARTESIAN_POINT ( 'NONE',  ( 37.56795767147776388, -285.5463622729420763, -258.9234100637174834 ) ) ;
#53369=CARTESIAN_POINT ( 'NONE',  ( 32.21273768267857207, -294.3096346340857963, -303.4690914269082782 ) ) ;
#53371=CARTESIAN_POINT ( 'NONE',  ( -78.18272752374834056, -289.9511686476623709, -330.9537812191658190 ) ) ;
#53374=CARTESIAN_POINT ( 'NONE',  ( -76.27077213493787156, -208.3870304207176787, -353.5830081017861062 ) ) ;
#53375=CARTESIAN_POINT ( 'NONE',  ( -91.42535153035444750, -286.8193444611971472, -216.5311411766099070 ) ) ;
#53376=CARTESIAN_POINT ( 'NONE',  ( 25.22466315766302358, -272.4094976428775681, -220.5068182859052968 ) ) ;
#53379=CARTESIAN_POINT ( 'NONE',  ( -37.55517273856889915, -281.9752483997886543, -343.6824025927108437 ) ) ;
#53380=CARTESIAN_POINT ( 'NONE',  ( -107.5585605960603601, -277.8143747117747466, -302.0397986969978774 ) ) ;
#53381=CARTESIAN_POINT ( 'NONE',  ( 31.70346837328679612, -283.1746699756419048, -241.5029626283152595 ) ) ;
#53382=CARTESIAN_POINT ( 'NONE',  ( 162.9489142668776935, 218.2876765797497001, -204.1083781671020176 ) ) ;
#53383=CARTESIAN_POINT ( 'NONE',  ( -3.172738037595201455, -281.1845061363202944, -338.7210183441566755 ) ) ;
#53384=CARTESIAN_POINT ( 'NONE',  ( 18.12945107263028888, -284.8727030029602361, -220.3940733625559005 ) ) ;
#53386=CARTESIAN_POINT ( 'NONE',  ( -72.82762065672925189, -299.3492022156100916, -203.1113437648492095 ) ) ;
#53387=CARTESIAN_POINT ( 'NONE',  ( -101.5183833719510460, -296.5682730717829827, -305.2801925593935835 ) ) ;
#53389=CARTESIAN_POINT ( 'NONE',  ( -41.60480967958189069, -290.6822996497886038, -196.9415307168669642 ) ) ;
#53390=CARTESIAN_POINT ( 'NONE',  ( -74.04089127183841867, -278.1779915879210989, -337.9518505832722894 ) ) ;
#53391=CARTESIAN_POINT ( 'NONE',  ( 35.58697269398483343, -275.4964550357007624, -266.1389709784803586 ) ) ;
#53392=CARTESIAN_POINT ( 'NONE',  ( 20.57773378394159636, -275.1547180929459273, -320.6485899078971897 ) ) ;
#53394=CARTESIAN_POINT ( 'NONE',  ( 2.977554037242769347, -272.5928393528377569, -207.0603478451820365 ) ) ;
#53395=CARTESIAN_POINT ( 'NONE',  ( -19.40782647434127384, -296.2512398688926396, -344.6919789385186164 ) ) ;
#53399=CARTESIAN_POINT ( 'NONE',  ( -107.6553532563122388, -285.9072115601640007, -249.4432875828630074 ) ) ;
#53400=CARTESIAN_POINT ( 'NONE',  ( -87.63385280214104966, -285.5028135864859564, -327.3933905286901336 ) ) ;
#53401=CARTESIAN_POINT ( 'NONE',  ( -105.3117712919072630, -283.5396761071032188, -297.4054939483576732 ) ) ;
#53402=CARTESIAN_POINT ( 'NONE',  ( 27.45956058052916759, -274.4301572430983924, -305.7841394545822595 ) ) ;
#53403=CARTESIAN_POINT ( 'NONE',  ( -6.722722166402029131, -284.5062970015063115, -338.0015672801819733 ) ) ;
#53404=CARTESIAN_POINT ( 'NONE',  ( -95.83504826728078285, -276.4073625159570611, -315.1856199629881985 ) ) ;
#53405=CARTESIAN_POINT ( 'NONE',  ( -36.44867144630563871, -278.1204099337319349, -343.6773115128813743 ) ) ;
#53407=CARTESIAN_POINT ( 'NONE',  ( -101.7614368603509689, -279.9072778027917821, -228.3809774570239881 ) ) ;
#53409=CARTESIAN_POINT ( 'NONE',  ( 27.79590931484954197, -281.5067918293200364, -229.3147521019760404 ) ) ;
#53413=CARTESIAN_POINT ( 'NONE',  ( 0.8777899896498234655, -288.4166783843363078, -204.9275593736371093 ) ) ;
#53414=CARTESIAN_POINT ( 'NONE',  ( -68.10612323592761186, -296.8347323899274102, -203.9685719074067265 ) ) ;
#53416=CARTESIAN_POINT ( 'NONE',  ( -68.02084141694460584, -288.7930953834055003, -340.8742591452510169 ) ) ;
#53417=CARTESIAN_POINT ( 'NONE',  ( 27.91345556135372874, -286.2628761704095837, -305.3948923158214370 ) ) ;
#53418=CARTESIAN_POINT ( 'NONE',  ( 25.46297528865467186, -285.6027102171243541, -232.0081824731794029 ) ) ;
#53419=CARTESIAN_POINT ( 'NONE',  ( -106.0621518300596335, -288.4275603878257925, -297.9846536262857057 ) ) ;
#53420=CARTESIAN_POINT ( 'NONE',  ( -74.93660346783462955, -286.7444044557256575, -207.3234011161567594 ) ) ;
#53421=CARTESIAN_POINT ( 'NONE',  ( -50.97472971357520777, -275.2262152481998783, -344.1116512024975691 ) ) ;
#53422=CARTESIAN_POINT ( 'NONE',  ( -31.90442097226439699, -287.3846355029374990, -346.4188938060080432 ) ) ;
#53423=CARTESIAN_POINT ( 'NONE',  ( 26.97010465818681624, -289.0344757514233152, -231.6735466715089728 ) ) ;
#53424=CARTESIAN_POINT ( 'NONE',  ( 22.41972231341030408, -284.9291229476012859, -224.7483309454040636 ) ) ;
#53425=CARTESIAN_POINT ( 'NONE',  ( 32.45922421033046845, -282.7882833614393121, -292.6902890776049162 ) ) ;
#53426=CARTESIAN_POINT ( 'NONE',  ( -98.36660046895637777, -291.9561389991337137, -314.2692624980895744 ) ) ;
#53429=CARTESIAN_POINT ( 'NONE',  ( -111.1982760520480866, -298.6763485988056459, -254.3469390481135122 ) ) ;
#53430=CARTESIAN_POINT ( 'NONE',  ( 13.45455668918196501, -279.9822231923999425, -217.6374746305969836 ) ) ;
#53431=CARTESIAN_POINT ( 'NONE',  ( 33.22803067003570732, -279.8829693749308944, -295.9096774006114288 ) ) ;
#53432=CARTESIAN_POINT ( 'NONE',  ( 23.89408600486299505, -293.3690069489301209, -316.7759573956556665 ) ) ;
#53433=CARTESIAN_POINT ( 'NONE',  ( -34.42000716631464030, -296.4891925136792565, -196.5619242977774661 ) ) ;
#53434=CARTESIAN_POINT ( 'NONE',  ( 34.55109611369488221, -280.0363492217385897, -255.0475872451824557 ) ) ;
#53435=CARTESIAN_POINT ( 'NONE',  ( 3.912214931269825779, -274.5716672616509868, -332.3242415992071415 ) ) ;
#53436=CARTESIAN_POINT ( 'NONE',  ( -38.33225214234089151, -296.3800019997042909, -343.8475948761143854 ) ) ;
#53438=CARTESIAN_POINT ( 'NONE',  ( -33.35986328002660883, -296.5810333359765991, -194.0554542064440966 ) ) ;
#53439=CARTESIAN_POINT ( 'NONE',  ( -14.11340134904579102, -292.9947589978014548, -342.7104106392622498 ) ) ;
#53441=CARTESIAN_POINT ( 'NONE',  ( -68.06359474647744889, -293.0659521925886111, -203.4776955545930548 ) ) ;
#53443=CARTESIAN_POINT ( 'NONE',  ( -9.675873773131842270, -293.2257645659203149, -202.5783187618469583 ) ) ;
#53446=CARTESIAN_POINT ( 'NONE',  ( -52.60954260745525346, -281.2667711915983091, -344.2067243930109726 ) ) ;
#53447=CARTESIAN_POINT ( 'NONE',  ( -0.7579505484019695150, -294.5520338759256447, -333.5902389464289399 ) ) ;
#53448=CIRCLE ( 'NONE', #12643, 2.500000000000008882 ) ;
#53449=CARTESIAN_POINT ( 'NONE',  ( -21.72598844115062633, -282.8572997399541578, -345.7610486755697252 ) ) ;
#53450=CARTESIAN_POINT ( 'NONE',  ( -5.572117537188898240, -282.3869056221775509, -201.8045149171525452 ) ) ;
#53451=CARTESIAN_POINT ( 'NONE',  ( -83.25986362943622510, -285.1093267773922548, -208.5106178740870462 ) ) ;
#53452=CARTESIAN_POINT ( 'NONE',  ( -67.27458302244387767, -289.6585701290007933, -201.7750337473001139 ) ) ;
#53453=CARTESIAN_POINT ( 'NONE',  ( 38.58615182004371036, -280.1342948216435502, -278.4643160311609904 ) ) ;
#53455=CARTESIAN_POINT ( 'NONE',  ( -4.358323734616576850, -285.1811774292669952, -204.6850922109212547 ) ) ;
#53456=CARTESIAN_POINT ( 'NONE',  ( -41.75656071397668256, -288.0268498034554909, -346.9379959245354712 ) ) ;
#53458=CARTESIAN_POINT ( 'NONE',  ( -3.956730053986134532, -296.2044205038557720, -336.1923221123482790 ) ) ;
#53459=CARTESIAN_POINT ( 'NONE',  ( -48.39070713424904824, -278.6152822394276996, -346.0223078551192657 ) ) ;
#53460=CARTESIAN_POINT ( 'NONE',  ( -71.35468269079774473, -293.5191821523822000, -337.6033950387694631 ) ) ;
#53461=CARTESIAN_POINT ( 'NONE',  ( -103.3871612008927912, -278.6410144359227843, -239.0961044356974412 ) ) ;
#53462=CARTESIAN_POINT ( 'NONE',  ( 21.30906725888254272, -293.0459835401329656, -220.4502198836788125 ) ) ;
#53464=CARTESIAN_POINT ( 'NONE',  ( -77.73168701141460701, -283.5941221504516534, -206.5021862943189603 ) ) ;
#53465=CARTESIAN_POINT ( 'NONE',  ( -89.90860393547966112, -279.7940334242371705, -323.9288789606204659 ) ) ;
#53466=CARTESIAN_POINT ( 'NONE',  ( -67.40271682585334645, -294.5151116790838159, -337.1561821627719269 ) ) ;
#53467=CARTESIAN_POINT ( 'NONE',  ( 50.67999509495882648, -297.1537971777466396, -195.3911227890569364 ) ) ;
#53471=CARTESIAN_POINT ( 'NONE',  ( 36.10835579765513614, -283.7045761038604610, -283.7346042300444537 ) ) ;
#53472=CARTESIAN_POINT ( 'NONE',  ( 34.96954119037157227, -292.9221476709713556, -259.9173245781427113 ) ) ;
#53474=CARTESIAN_POINT ( 'NONE',  ( 90.38368222445549804, -297.2649936051623740, -200.4191791630918829 ) ) ;
#53475=CARTESIAN_POINT ( 'NONE',  ( -109.9459350855805582, -272.0671327394398986, -245.2059219683897595 ) ) ;
#53478=CARTESIAN_POINT ( 'NONE',  ( -2.013457625617498525, -289.9093712104926794, -338.2228417725291933 ) ) ;
#53479=CARTESIAN_POINT ( 'NONE',  ( -86.73094157181898822, -289.5950122741907649, -324.1856509083503397 ) ) ;
#53480=CARTESIAN_POINT ( 'NONE',  ( -85.95594508165648051, -280.8839895215666047, -214.9773393255055680 ) ) ;
#53481=CARTESIAN_POINT ( 'NONE',  ( -82.58097277338399067, -299.1849767516310976, -211.7181474457664763 ) ) ;
#53483=CARTESIAN_POINT ( 'NONE',  ( -89.74639259215807385, -278.0876277746680785, -218.8996260977656618 ) ) ;
#53485=CARTESIAN_POINT ( 'NONE',  ( -87.44527960819715418, -297.0423475492891043, -211.8496367412311372 ) ) ;
#53486=CARTESIAN_POINT ( 'NONE',  ( -38.95278486730700962, -293.9519368886932398, -195.9385501220022263 ) ) ;
#53487=CARTESIAN_POINT ( 'NONE',  ( 33.71294247884864603, -295.5046525977163583, -297.8870726060117704 ) ) ;
#53489=CARTESIAN_POINT ( 'NONE',  ( -110.2235594616041112, -291.1207647228275732, -276.6469173351887321 ) ) ;
#53491=ORIENTED_EDGE ( 'NONE', *, *, #37667, .F. ) ;
#53492=CARTESIAN_POINT ( 'NONE',  ( 36.85714900344527933, -291.4961551925204617, -254.9730681394802900 ) ) ;
#53493=CARTESIAN_POINT ( 'NONE',  ( -96.11481449953545564, -296.8262765204489142, -227.0063217345130511 ) ) ;
#53496=CARTESIAN_POINT ( 'NONE',  ( -110.5722806347883989, -292.3437203761134811, -248.9137444395219916 ) ) ;
#53497=CARTESIAN_POINT ( 'NONE',  ( -55.56934967048406548, -285.7662352645559736, -350.3683826091709648 ) ) ;
#53498=CARTESIAN_POINT ( 'NONE',  ( 20.92705608575735710, -288.9044396565371358, -223.3857331067162875 ) ) ;
#53499=CARTESIAN_POINT ( 'NONE',  ( 14.79167515850976677, -272.7886193602478215, -216.6755556202300852 ) ) ;
#53500=CARTESIAN_POINT ( 'NONE',  ( 34.99148296292155891, -277.7004603218841225, -287.9996778581713102 ) ) ;
#53501=CARTESIAN_POINT ( 'NONE',  ( -68.37974481075222855, -289.7210671076290964, -202.6865360694132505 ) ) ;
#53502=CARTESIAN_POINT ( 'NONE',  ( -9.340007922585357392, -282.2747235136142194, -199.9607577945520802 ) ) ;
#53504=CARTESIAN_POINT ( 'NONE',  ( 22.66370920053164895, -281.4818807707252972, -312.1132858258388296 ) ) ;
#53505=CARTESIAN_POINT ( 'NONE',  ( -113.9226030530051759, -279.5802657903545878, -274.4669450821897385 ) ) ;
#53506=CARTESIAN_POINT ( 'NONE',  ( -8.993714353747773060, -279.2097266652032204, -199.1965170824571487 ) ) ;
#53507=CARTESIAN_POINT ( 'NONE',  ( -83.89489645444281507, -218.2138212151350274, -349.1709152291787177 ) ) ;
#53508=CARTESIAN_POINT ( 'NONE',  ( 24.28379887806177351, -275.8829143854081281, -224.5886580769461318 ) ) ;
#53510=CARTESIAN_POINT ( 'NONE',  ( -13.29945240308443921, -275.8789925598883883, -197.9409683283515164 ) ) ;
#53511=CARTESIAN_POINT ( 'NONE',  ( 30.91033621190086578, -278.2662352645559167, -285.9065529553535612 ) ) ;
#53513=EDGE_LOOP ( 'NONE', ( #18409, #4163 ) ) ;
#53516=CARTESIAN_POINT ( 'NONE',  ( -71.30380130000267513, -290.5912667105385481, -335.3429969690661778 ) ) ;
#53517=CARTESIAN_POINT ( 'NONE',  ( -73.91959465289349396, -291.2911794191204535, -336.9795121209891704 ) ) ;
#53518=CARTESIAN_POINT ( 'NONE',  ( -69.05432617537894657, -290.9723524827647338, -204.4822673447438603 ) ) ;
#53519=CARTESIAN_POINT ( 'NONE',  ( -54.94443600254491145, -285.3393235402896266, -195.4633837525568083 ) ) ;
#53521=CARTESIAN_POINT ( 'NONE',  ( -0.8742267934148434394, -280.9591169538946360, -334.5215715681413258 ) ) ;
#53522=CARTESIAN_POINT ( 'NONE',  ( 35.98294356602544752, -289.5639908884725173, -282.0337551559471763 ) ) ;
#53523=CARTESIAN_POINT ( 'NONE',  ( -93.96713309904129119, -282.3691525895853829, -317.5232648284304560 ) ) ;
#53524=CARTESIAN_POINT ( 'NONE',  ( 28.21375808265830187, -282.4179217206897192, -237.0259640415451656 ) ) ;
#53525=CARTESIAN_POINT ( 'NONE',  ( 34.85528321835723631, -288.8255783650404283, -296.6006222123673979 ) ) ;
#53527=CARTESIAN_POINT ( 'NONE',  ( -108.5448247499395364, -278.8279534006231302, -286.7904078305830353 ) ) ;
#53528=CARTESIAN_POINT ( 'NONE',  ( 35.91178520937113205, -292.0643128753050064, -247.9571985800041318 ) ) ;
#53529=CARTESIAN_POINT ( 'NONE',  ( 26.99695284087917102, -287.8019280925874455, -228.3528264855224847 ) ) ;
#53530=CARTESIAN_POINT ( 'NONE',  ( -30.89526345505026583, -286.6238772477501584, -193.6799112136753820 ) ) ;
#53531=CARTESIAN_POINT ( 'NONE',  ( -92.55773708211756912, -284.0382644706018027, -318.1314672899030143 ) ) ;
#53534=CARTESIAN_POINT ( 'NONE',  ( -39.20544239675091802, -293.8894398156688226, -194.6064151012685954 ) ) ;
#53536=CARTESIAN_POINT ( 'NONE',  ( -2.208946272988375537, -293.2817535578410570, -338.3242541719755536 ) ) ;
#53537=AXIS2_PLACEMENT_3D ( 'NONE', #65653, #52792, #23468 ) ;
#53538=CARTESIAN_POINT ( 'NONE',  ( -4.972844100947378720, -275.6739725832372869, -336.0687780714280848 ) ) ;
#53539=CARTESIAN_POINT ( 'NONE',  ( -36.17796258691097222, -297.4149543911442493, -193.4631747941452602 ) ) ;
#53540=CARTESIAN_POINT ( 'NONE',  ( -103.0187801208346912, -289.4830747739144954, -236.8232416528182114 ) ) ;
#53541=CARTESIAN_POINT ( 'NONE',  ( -31.54504799889173228, -293.2179654760569747, -344.1979205509059625 ) ) ;
#53542=CARTESIAN_POINT ( 'NONE',  ( -64.23129220876163004, -292.8984199429332875, -202.0534374675834499 ) ) ;
#53543=CARTESIAN_POINT ( 'NONE',  ( 0.05496061932472129374, -293.6423373684970670, -207.3078402041178947 ) ) ;
#53546=CARTESIAN_POINT ( 'NONE',  ( -66.24363585937848597, -293.4294178778324067, -339.7630703501282596 ) ) ;
#53547=CARTESIAN_POINT ( 'NONE',  ( -110.7090265421391848, -298.7529277821208780, -254.7365277776543167 ) ) ;
#53548=CARTESIAN_POINT ( 'NONE',  ( 8.135397859867781634, -289.3536494916072570, -327.7653164872236857 ) ) ;
#53549=CARTESIAN_POINT ( 'NONE',  ( 35.65191476376229929, -277.7713883502986505, -289.0784626392904784 ) ) ;
#53550=CARTESIAN_POINT ( 'NONE',  ( -38.55414350765858700, -275.8619687045352293, -346.9544512512505889 ) ) ;
#53552=CARTESIAN_POINT ( 'NONE',  ( -15.79795347058474775, -273.6721948758317922, -196.4872904889921017 ) ) ;
#53553=CARTESIAN_POINT ( 'NONE',  ( 31.35970305550844017, -279.2549865558309534, -241.7004934963151470 ) ) ;
#53554=CARTESIAN_POINT ( 'NONE',  ( -69.97707815762707639, -275.8746695921522019, -339.2330318381748384 ) ) ;
#53555=CARTESIAN_POINT ( 'NONE',  ( -108.9538164803419704, -295.4534563665711175, -253.8399717972104099 ) ) ;
#53557=CARTESIAN_POINT ( 'NONE',  ( 9.047129706206952449, -299.4503132403827976, -197.1931170228812391 ) ) ;
#53559=CARTESIAN_POINT ( 'NONE',  ( 21.11292379528279994, -286.2244386629721475, -317.9362664230023370 ) ) ;
#53560=CARTESIAN_POINT ( 'NONE',  ( -8.968870243490044913, -274.2670615027375902, -203.0466486310713208 ) ) ;
#53561=CARTESIAN_POINT ( 'NONE',  ( 34.04233153705654047, -287.9202441031945909, -299.3704214840180953 ) ) ;
#53562=CARTESIAN_POINT ( 'NONE',  ( -36.58718554504064713, -300.0414395763572770, -195.0056563871800961 ) ) ;
#53563=CARTESIAN_POINT ( 'NONE',  ( -105.3749723034196961, -294.9635199266085124, -239.0675551975072892 ) ) ;
#53564=CARTESIAN_POINT ( 'NONE',  ( -70.40991195299049821, -282.6741159565261228, -339.7344152150485570 ) ) ;
#53565=CARTESIAN_POINT ( 'NONE',  ( -47.57981157014602758, -281.1820066073696580, -344.7108298921560845 ) ) ;
#53567=CARTESIAN_POINT ( 'NONE',  ( -110.5198391537857106, -289.2645747620837255, -276.6487320007701101 ) ) ;
#53568=CARTESIAN_POINT ( 'NONE',  ( -53.98933082536719041, -281.4075750347531084, -342.7585545661566471 ) ) ;
#53571=CARTESIAN_POINT ( 'NONE',  ( -82.92494501057666412, -289.4288575006773385, -210.7373074863700424 ) ) ;
#53572=CARTESIAN_POINT ( 'NONE',  ( -85.78032882165403805, -274.8875901406511275, -214.7556516067056123 ) ) ;
#53573=CARTESIAN_POINT ( 'NONE',  ( -35.89124574053997208, -284.2394436499364474, -346.9633628334771629 ) ) ;
#53574=CARTESIAN_POINT ( 'NONE',  ( -87.06992988784264753, -271.4462442710271830, -213.4020553476225075 ) ) ;
#53575=CARTESIAN_POINT ( 'NONE',  ( -42.93291624435025966, -283.1245427785490847, -343.1967683786787688 ) ) ;
#53576=CARTESIAN_POINT ( 'NONE',  ( 28.56624908000236474, -277.4190832319022775, -303.2100869034903781 ) ) ;
#53577=CARTESIAN_POINT ( 'NONE',  ( 13.85160733464844895, -277.1148272192308468, -322.6987577167236623 ) ) ;
#53578=CARTESIAN_POINT ( 'NONE',  ( 20.09522755024080709, -284.2189616304831361, -318.5897400956937986 ) ) ;
#53582=CARTESIAN_POINT ( 'NONE',  ( 39.71162213157823118, -293.3848591304944762, -270.3120772472653357 ) ) ;
#53583=CARTESIAN_POINT ( 'NONE',  ( 26.34113441162241287, -289.0073260160251607, -231.4208639232660403 ) ) ;
#53585=CARTESIAN_POINT ( 'NONE',  ( -2.602324593224659921, -283.9809262143061233, -198.2974183793908196 ) ) ;
#53586=CARTESIAN_POINT ( 'NONE',  ( -75.26541960986445190, -276.7415813065929342, -337.1888840775224594 ) ) ;
#53588=CARTESIAN_POINT ( 'NONE',  ( -47.61515047640244092, -290.3236410794101516, -194.8036015930892120 ) ) ;
#53589=CIRCLE ( 'NONE', #91354, 2.939656322713313230 ) ;
#53590=CARTESIAN_POINT ( 'NONE',  ( -75.09174444536915871, -287.0593998682140864, -207.0709773090904378 ) ) ;
#53591=CARTESIAN_POINT ( 'NONE',  ( 1.420975651464791989, -278.2871051671716032, -333.4723521498562491 ) ) ;
#53592=CARTESIAN_POINT ( 'NONE',  ( -0.01998350143177623009, -287.9639790831113260, -203.6701362938990769 ) ) ;
#53593=CARTESIAN_POINT ( 'NONE',  ( 31.15105857745839302, -283.9542864903835380, -301.0459345715297559 ) ) ;
#53594=CARTESIAN_POINT ( 'NONE',  ( 34.18504415190763268, -276.0821638689352540, -299.0167176371553523 ) ) ;
#53595=CARTESIAN_POINT ( 'NONE',  ( -99.65101279177115146, -277.7850142952611350, -315.6223448987266806 ) ) ;
#53596=CARTESIAN_POINT ( 'NONE',  ( -66.15218053224842265, -299.5922466657734731, -201.7224232228427070 ) ) ;
#53599=CARTESIAN_POINT ( 'NONE',  ( 31.95455697924148097, -283.6233781216988064, -236.9535640164627637 ) ) ;
#53600=CARTESIAN_POINT ( 'NONE',  ( -45.96538147938693442, -296.0834832649001100, -195.0886954144488925 ) ) ;
#53603=CARTESIAN_POINT ( 'NONE',  ( -96.14626180808231481, -277.4523749078908281, -313.7411953049549425 ) ) ;
#53604=CARTESIAN_POINT ( 'NONE',  ( -92.89483106924163280, -274.4819131641421563, -217.5986463183466242 ) ) ;
#53605=CARTESIAN_POINT ( 'NONE',  ( 22.69880531111737909, -279.9683447281902886, -222.5076124784726233 ) ) ;
#53606=CARTESIAN_POINT ( 'NONE',  ( 11.79022208728040866, -288.5053483433746919, -214.9386120569807588 ) ) ;
#53607=CARTESIAN_POINT ( 'NONE',  ( -53.12674506964882681, -296.7709695311993983, -345.0713127741260564 ) ) ;
#53608=CARTESIAN_POINT ( 'NONE',  ( -105.5968944431117791, -297.3057655846544662, -305.2520074802090448 ) ) ;
#53609=CARTESIAN_POINT ( 'NONE',  ( -44.50032219989088134, -293.9616707823158777, -195.8188722004524891 ) ) ;
#53610=CARTESIAN_POINT ( 'NONE',  ( 36.85386958613226227, -279.4215622442948757, -260.2257207562183225 ) ) ;
#53611=CARTESIAN_POINT ( 'NONE',  ( 14.31715667453972252, -282.7047712181081351, -216.6919510423215058 ) ) ;
#53612=CARTESIAN_POINT ( 'NONE',  ( -37.12127030869519473, -296.1347879267162284, -195.9182775452011072 ) ) ;
#53613=CARTESIAN_POINT ( 'NONE',  ( -91.84712396182010252, -285.4140936960852741, -323.6114624651132772 ) ) ;
#53614=AXIS2_PLACEMENT_3D ( 'NONE', #79126, #14273, #72038 ) ;
#53615=CARTESIAN_POINT ( 'NONE',  ( 27.29655540154662319, -286.9432364762299130, -305.0541176609947911 ) ) ;
#53616=CARTESIAN_POINT ( 'NONE',  ( 19.09100179000933650, -280.1882620950287901, -218.1245126101040341 ) ) ;
#53617=CARTESIAN_POINT ( 'NONE',  ( -88.39795797536243072, -231.3176004196124893, -347.5402749026013680 ) ) ;
#53619=CARTESIAN_POINT ( 'NONE',  ( 20.35997111928813652, -286.5887492913134338, -225.6106473467234821 ) ) ;
#53621=CARTESIAN_POINT ( 'NONE',  ( -74.11562602863301663, -284.6083464732569723, -337.7194813484299516 ) ) ;
#53622=CARTESIAN_POINT ( 'NONE',  ( 5.185615645001697693, -274.9781837824386912, -210.9394231862558229 ) ) ;
#53623=CARTESIAN_POINT ( 'NONE',  ( 25.22968011714511150, -285.7590275954245840, -226.1476479710968022 ) ) ;
#53624=CARTESIAN_POINT ( 'NONE',  ( -56.09981911720402081, -290.7364901304574119, -195.9449417016573989 ) ) ;
#53625=CARTESIAN_POINT ( 'NONE',  ( 21.78179697170708451, -281.8331784073755557, -221.3995789486758383 ) ) ;
#53627=CARTESIAN_POINT ( 'NONE',  ( -33.96549430379967305, -281.6140185880648232, -194.1291759367820475 ) ) ;
#53628=CARTESIAN_POINT ( 'NONE',  ( 36.57822742821990403, -281.6153989051564963, -248.8292581370362768 ) ) ;
#53629=CARTESIAN_POINT ( 'NONE',  ( -82.08285599513421005, -288.9094976428775681, -214.2051214447836571 ) ) ;
#53630=CARTESIAN_POINT ( 'NONE',  ( -21.48569620681853465, -108.6157210391733514, -362.8212015391057434 ) ) ;
#53632=CARTESIAN_POINT ( 'NONE',  ( -7.996861572670578511, -278.6670339975016759, -339.2147363236462638 ) ) ;
#53633=CARTESIAN_POINT ( 'NONE',  ( 184.4162654869148525, 263.6987771649366437, -153.0423760906433870 ) ) ;
#53634=CARTESIAN_POINT ( 'NONE',  ( 23.12995493623812138, -280.1712441473311515, -314.1440003197535020 ) ) ;
#53635=CARTESIAN_POINT ( 'NONE',  ( -98.52834922945847040, -296.4554326089141796, -230.2684471384125970 ) ) ;
#53636=CARTESIAN_POINT ( 'NONE',  ( -16.63714383042016820, -291.8203596798856552, -196.2608598751364184 ) ) ;
#53637=CARTESIAN_POINT ( 'NONE',  ( -109.4300717440919186, -269.0112169713418098, -295.3470023912256579 ) ) ;
#53638=CARTESIAN_POINT ( 'NONE',  ( -33.35434752022145943, -296.6758848936784716, -193.9512867474840334 ) ) ;
#53639=CARTESIAN_POINT ( 'NONE',  ( 33.04264522483112643, -285.6605388598512718, -248.1267844340309807 ) ) ;
#53640=CARTESIAN_POINT ( 'NONE',  ( 17.08052670803324702, -296.1261134211091530, -320.8495989157309509 ) ) ;
#53641=CARTESIAN_POINT ( 'NONE',  ( -69.00245828154172045, -286.9420105298405588, -204.0234830594493474 ) ) ;
#53643=CARTESIAN_POINT ( 'NONE',  ( -4.715066979952252879, -293.4127470249062526, -200.8749825059219063 ) ) ;
#53644=CARTESIAN_POINT ( 'NONE',  ( -103.0652842761183763, -284.6114456443505674, -302.3896500212662204 ) ) ;
#53645=CARTESIAN_POINT ( 'NONE',  ( -100.4149617698935231, -295.9242530994878848, -226.8665603547654541 ) ) ;
#53646=CARTESIAN_POINT ( 'NONE',  ( -27.87913822265212005, -292.9720822856205018, -194.0539093926565499 ) ) ;
#53647=CARTESIAN_POINT ( 'NONE',  ( -99.98459185586217757, -291.6366128526522630, -225.6912733521691052 ) ) ;
#53648=CARTESIAN_POINT ( 'NONE',  ( -74.71407828275975760, -289.7312495634576521, -333.0839009449283594 ) ) ;
#53651=CARTESIAN_POINT ( 'NONE',  ( -35.53294294358471461, -299.9349756489463061, -194.5957445222843205 ) ) ;
#53652=CARTESIAN_POINT ( 'NONE',  ( -94.77853345212247405, -272.0369759094540427, -219.6756279791674444 ) ) ;
#53653=CARTESIAN_POINT ( 'NONE',  ( -26.72045869150398545, -281.9726197832043795, -342.8735899217874135 ) ) ;
#53654=EDGE_LOOP ( 'NONE', ( #90824, #74321 ) ) ;
#53656=CARTESIAN_POINT ( 'NONE',  ( -72.81788955465673041, -277.0169313983098505, -338.6470847179453472 ) ) ;
#53657=CARTESIAN_POINT ( 'NONE',  ( -96.91522037678048207, -271.5564133648870211, -226.7166739224035723 ) ) ;
#53658=CARTESIAN_POINT ( 'NONE',  ( -79.78008251369473669, -281.3319343954994451, -209.4525867362486338 ) ) ;
#53659=CARTESIAN_POINT ( 'NONE',  ( -40.58301655547638376, -275.2328944556943497, -344.5382005577882296 ) ) ;
#53660=CARTESIAN_POINT ( 'NONE',  ( -110.6095666347328859, -297.8143495713083553, -266.0079304797559985 ) ) ;
#53661=CARTESIAN_POINT ( 'NONE',  ( -73.00925116881927579, -298.6472176279314681, -206.3138551465477804 ) ) ;
#53662=CARTESIAN_POINT ( 'NONE',  ( -93.09151525179012765, -298.8684963103057726, -218.3380175319154830 ) ) ;
#53663=CARTESIAN_POINT ( 'NONE',  ( -66.86743861542525735, -271.6872685160179799, -201.0311996820545630 ) ) ;
#53664=CARTESIAN_POINT ( 'NONE',  ( 22.66687361824671143, -293.6222339179165601, -228.5914461338662136 ) ) ;
#53665=CARTESIAN_POINT ( 'NONE',  ( -49.77052455606787618, -290.4653785447424639, -197.7773230103978221 ) ) ;
#53667=CARTESIAN_POINT ( 'NONE',  ( 38.66583559413955129, -275.8940849991554387, -258.3438715168978206 ) ) ;
#53668=CARTESIAN_POINT ( 'NONE',  ( -83.19223263293157800, -273.5702973329051702, -213.5568164420559754 ) ) ;
#53669=CARTESIAN_POINT ( 'NONE',  ( 27.87580258256984322, -280.7641343703041343, -310.4611761175884794 ) ) ;
#53672=CARTESIAN_POINT ( 'NONE',  ( -110.5520817729917837, -283.7422173350662433, -270.9003088089290259 ) ) ;
#53674=CARTESIAN_POINT ( 'NONE',  ( -58.00775052530494236, -281.3182150687318881, -342.6852303894619354 ) ) ;
#53675=CARTESIAN_POINT ( 'NONE',  ( 35.42702256844754061, -273.9823608123143117, -259.3177322871711681 ) ) ;
#53676=CARTESIAN_POINT ( 'NONE',  ( -48.54107235922690933, -281.9098679950072892, -196.1503743120290721 ) ) ;
#53679=CARTESIAN_POINT ( 'NONE',  ( -2.900705312295462690, -272.8994809571926226, -202.3740844392764302 ) ) ;
#53681=CARTESIAN_POINT ( 'NONE',  ( -112.3821156058396724, -280.6081071499053223, -266.0062966425177819 ) ) ;
#53683=CARTESIAN_POINT ( 'NONE',  ( -91.38637037264089713, -285.7340677702808875, -323.1672522424606200 ) ) ;
#53686=CARTESIAN_POINT ( 'NONE',  ( -104.3669543607152406, -288.9978052692231927, -236.5926037552136165 ) ) ;
#53689=CARTESIAN_POINT ( 'NONE',  ( -109.7571711225060085, -295.1901049508429651, -282.3248158213936563 ) ) ;
#53690=CARTESIAN_POINT ( 'NONE',  ( 6.556285905353787413, -286.5883643556964557, -330.2902834661385896 ) ) ;
#53692=CARTESIAN_POINT ( 'NONE',  ( -105.5265176478331028, -294.9635199286505554, -238.9979103698759388 ) ) ;
#53693=CARTESIAN_POINT ( 'NONE',  ( 23.32212481994681141, -285.4090837977557840, -224.0513729359206820 ) ) ;
#53694=CARTESIAN_POINT ( 'NONE',  ( 35.11584125794944811, -282.9685739567360656, -256.2823163011307770 ) ) ;
#53695=CARTESIAN_POINT ( 'NONE',  ( -49.94776518472127691, -281.4505837710136689, -345.3479975934111508 ) ) ;
#53696=CARTESIAN_POINT ( 'NONE',  ( -15.85164981939449547, -288.7664298321241176, -340.1791045327702818 ) ) ;
#53697=CARTESIAN_POINT ( 'NONE',  ( 34.64616932668712934, -282.5277066901281842, -283.4831276537292410 ) ) ;
#53699=CARTESIAN_POINT ( 'NONE',  ( -0.07178170301374783846, -290.5391178371183400, -335.9132986364966769 ) ) ;
#53700=CARTESIAN_POINT ( 'NONE',  ( -75.78174656667668785, -297.7208338461131234, -203.5813900550990354 ) ) ;
#53701=CARTESIAN_POINT ( 'NONE',  ( -67.53564237597846898, -273.6668407948344566, -199.5280335408201040 ) ) ;
#53702=CARTESIAN_POINT ( 'NONE',  ( -25.16507031956652085, -294.1879209930351635, -196.6635469330276180 ) ) ;
#53704=CARTESIAN_POINT ( 'NONE',  ( -114.2704648735229114, -287.0519495502703080, -270.3937649182068981 ) ) ;
#53706=CARTESIAN_POINT ( 'NONE',  ( 20.30776064926366686, -274.2169863109052699, -318.5956295083899477 ) ) ;
#53708=CARTESIAN_POINT ( 'NONE',  ( -112.9782036321411169, -295.0689229741468580, -261.1112665015822927 ) ) ;
#53709=CARTESIAN_POINT ( 'NONE',  ( -109.9625467149489424, -291.9808278973164306, -283.5008690240114220 ) ) ;
#53710=CARTESIAN_POINT ( 'NONE',  ( -34.02776938650374916, -273.4435175781427461, -197.3343384325569616 ) ) ;
#53711=CARTESIAN_POINT ( 'NONE',  ( -110.9983512697878041, -292.0252275883647144, -273.9619563567424052 ) ) ;
#53712=CARTESIAN_POINT ( 'NONE',  ( -57.73191080878844161, -292.7236976606802727, -199.9685503581490309 ) ) ;
#53713=CARTESIAN_POINT ( 'NONE',  ( -53.89479585623762148, -285.0275496555290715, -342.5524618780006563 ) ) ;
#53714=CARTESIAN_POINT ( 'NONE',  ( -97.01487597653033390, -292.6215975127229285, -222.6356700551351082 ) ) ;
#53715=CARTESIAN_POINT ( 'NONE',  ( -76.92852493151174542, -292.8491664829326737, -204.8310765265192686 ) ) ;
#53716=CARTESIAN_POINT ( 'NONE',  ( -0.7597893167630116462, -294.3853807310752586, -333.5913030011353158 ) ) ;
#53717=CARTESIAN_POINT ( 'NONE',  ( 26.64409949748151618, -289.0275910412937037, -231.2354474640682440 ) ) ;
#53718=CARTESIAN_POINT ( 'NONE',  ( 26.27941828610472541, -281.1457015852035966, -226.8935177391313971 ) ) ;
#53719=CARTESIAN_POINT ( 'NONE',  ( -71.44638058470263786, -293.5789106112503077, -337.7865210031841343 ) ) ;
#53720=CARTESIAN_POINT ( 'NONE',  ( -108.2279708245690983, -284.0012034924757245, -300.5663936039224495 ) ) ;
#53721=CARTESIAN_POINT ( 'NONE',  ( 36.99424976649718388, -277.6195602777492581, -277.1444323805264958 ) ) ;
#53723=CARTESIAN_POINT ( 'NONE',  ( 4.096446069770744991, -284.6098817895948514, -207.7862039460869141 ) ) ;
#53724=CARTESIAN_POINT ( 'NONE',  ( -56.63277164091257276, -275.4376916734761949, -343.6830209935733365 ) ) ;
#53726=CARTESIAN_POINT ( 'NONE',  ( -29.44422744186875462, -282.4572117539385090, -343.0451161892349319 ) ) ;
#53727=CARTESIAN_POINT ( 'NONE',  ( -95.61379339938980593, -280.4315221119219927, -220.6180146963801860 ) ) ;
#53728=CARTESIAN_POINT ( 'NONE',  ( 18.18959880444806032, -285.8832565510972472, -217.2835471050289584 ) ) ;
#53729=CARTESIAN_POINT ( 'NONE',  ( 31.53671491733354415, -295.6712145854739902, -297.5890486515670545 ) ) ;
#53730=CARTESIAN_POINT ( 'NONE',  ( 36.81805767896555892, -277.3742741319258016, -287.9322581230598530 ) ) ;
#53731=CARTESIAN_POINT ( 'NONE',  ( 33.73238483501313567, -277.2304729315533223, -298.8196200745537681 ) ) ;
#53732=CARTESIAN_POINT ( 'NONE',  ( -103.1319309202313264, -277.9561026858974628, -302.1110714914964888 ) ) ;
#53733=CARTESIAN_POINT ( 'NONE',  ( -102.1582459998145112, -275.0293437238689762, -233.2346628275964235 ) ) ;
#53734=CARTESIAN_POINT ( 'NONE',  ( 19.17715791613656862, -284.8699592250636101, -221.3137213729414725 ) ) ;
#53735=CARTESIAN_POINT ( 'NONE',  ( -34.85957701735164704, -294.6884888296338545, -347.2999466483493620 ) ) ;
#53736=CARTESIAN_POINT ( 'NONE',  ( -91.02035993566803995, -291.3987747300134288, -324.5189800521484926 ) ) ;
#53737=CARTESIAN_POINT ( 'NONE',  ( 22.06323377204606473, -291.8738325072574185, -227.3830450239286165 ) ) ;
#53739=CARTESIAN_POINT ( 'NONE',  ( -28.09946630545501023, -291.8392725812647086, -197.8764635893611796 ) ) ;
#53741=CARTESIAN_POINT ( 'NONE',  ( -84.96193311972864137, -290.7710090362177766, -330.5438033894057526 ) ) ;
#53742=CARTESIAN_POINT ( 'NONE',  ( -59.77278706339543390, -280.4053062131053480, -200.7323170001139374 ) ) ;
#53743=CARTESIAN_POINT ( 'NONE',  ( -89.38839166277168147, -296.2602100345200142, -213.9630494963244018 ) ) ;
#53744=CARTESIAN_POINT ( 'NONE',  ( 26.26837592287659362, -287.6328268496965848, -227.1279820120310546 ) ) ;
#53745=CARTESIAN_POINT ( 'NONE',  ( 37.69806526446761552, -287.6699898611338426, -253.1335338145305798 ) ) ;
#53746=CARTESIAN_POINT ( 'NONE',  ( -106.5537135154276172, -285.1964224836257813, -246.9264936854656014 ) ) ;
#53747=CARTESIAN_POINT ( 'NONE',  ( 193.7935517605804989, 279.2504548556453869, -125.8485263907484750 ) ) ;
#53748=CARTESIAN_POINT ( 'NONE',  ( 183.4698700144519989, 263.1936897402629825, -152.3596953817753672 ) ) ;
#53749=CARTESIAN_POINT ( 'NONE',  ( -12.93242418913286329, -92.20420405495083571, -356.2274306187722459 ) ) ;
#53750=CARTESIAN_POINT ( 'NONE',  ( 15.70794271834726530, -275.4740003981351606, -320.7430306185804056 ) ) ;
#53751=CARTESIAN_POINT ( 'NONE',  ( 17.65807200446980474, -275.1618888144814150, -318.8491255472634407 ) ) ;
#53752=CARTESIAN_POINT ( 'NONE',  ( -108.0563970603190000, -272.6079619551429118, -239.8096252077025952 ) ) ;
#53753=CARTESIAN_POINT ( 'NONE',  ( 46.50877722536523606, 10.63732441549002949, -329.0452962795232565 ) ) ;
#53754=CARTESIAN_POINT ( 'NONE',  ( -54.04003407429214434, -275.9469056853669144, -345.0777433922604018 ) ) ;
#53756=CARTESIAN_POINT ( 'NONE',  ( -37.26166180947142692, -289.5434718961854514, -343.4226128738837929 ) ) ;
#53757=CARTESIAN_POINT ( 'NONE',  ( -108.7423483825970720, -297.7175025026989488, -241.8260749796072275 ) ) ;
#53758=CARTESIAN_POINT ( 'NONE',  ( -51.79520661962206418, -298.3644645993396693, -194.7381567659673181 ) ) ;
#53759=CARTESIAN_POINT ( 'NONE',  ( -26.20531350542740512, -295.0731009240769254, -342.5066715356343821 ) ) ;
#53761=CARTESIAN_POINT ( 'NONE',  ( -103.6990812841965663, -279.9957073324142698, -306.4999082441668179 ) ) ;
#53762=CARTESIAN_POINT ( 'NONE',  ( 39.55810021491750916, -281.0903305709754818, -272.7998902695285324 ) ) ;
#53763=CARTESIAN_POINT ( 'NONE',  ( -103.6553095478218296, -280.0537396808990707, -238.9890532526910931 ) ) ;
#53764=CARTESIAN_POINT ( 'NONE',  ( -56.64468163391967437, -279.0576661757560260, -343.9094473348219481 ) ) ;
#53765=CARTESIAN_POINT ( 'NONE',  ( -88.52261674738612385, -295.8923777569148683, -217.4138278520737515 ) ) ;
#53767=CARTESIAN_POINT ( 'NONE',  ( -97.99479180768965136, -279.2841262416791324, -229.6486716486747355 ) ) ;
#53768=CARTESIAN_POINT ( 'NONE',  ( -63.51172613709964310, -274.5224141247678062, -198.1164741741325486 ) ) ;
#53769=CARTESIAN_POINT ( 'NONE',  ( 37.33987683817696990, -286.4468324700234234, -287.0329228604045397 ) ) ;
#53770=CARTESIAN_POINT ( 'NONE',  ( -8.484289576188103865, -276.4298878468243288, -201.0799179885277681 ) ) ;
#53771=CARTESIAN_POINT ( 'NONE',  ( 27.14175265579480367, -274.6694386990668590, -311.4532224839380774 ) ) ;
#53773=CARTESIAN_POINT ( 'NONE',  ( -107.8842409054083618, -289.4913365489192074, -289.9476935304697349 ) ) ;
#53774=CARTESIAN_POINT ( 'NONE',  ( -99.71067791559507043, -283.3025203649021933, -315.4325958904153140 ) ) ;
#53775=CARTESIAN_POINT ( 'NONE',  ( 36.71648401343644252, -279.8048610585829579, -271.3493513211785171 ) ) ;
#53776=CARTESIAN_POINT ( 'NONE',  ( 13.75720791185352709, -279.3598837390550216, -217.3346685025056786 ) ) ;
#53777=CARTESIAN_POINT ( 'NONE',  ( -84.54243050674024573, -283.4765621198396843, -212.7319753606611528 ) ) ;
#53778=CARTESIAN_POINT ( 'NONE',  ( -36.66223718241194263, -291.0438312036703792, -345.3706420096863781 ) ) ;
#53779=CARTESIAN_POINT ( 'NONE',  ( -110.5558063710717960, -279.8251882676347009, -265.1818177385400759 ) ) ;
#53781=CARTESIAN_POINT ( 'NONE',  ( 31.65922809037965990, -280.3717877619147885, -302.8166510391656630 ) ) ;
#53782=CARTESIAN_POINT ( 'NONE',  ( 37.71021853838445281, -295.5513509988829242, -270.2858652379441082 ) ) ;
#53783=CARTESIAN_POINT ( 'NONE',  ( -99.40817597146521223, -277.3798445903617562, -226.5236158756072200 ) ) ;
#53784=CARTESIAN_POINT ( 'NONE',  ( -109.3443127197655116, -286.2743845897448978, -291.9847375159998819 ) ) ;
#53785=CARTESIAN_POINT ( 'NONE',  ( -33.63493029267698375, -294.0186186291767285, -194.8920908453042102 ) ) ;
#53786=CARTESIAN_POINT ( 'NONE',  ( 36.62618604559104085, -287.0111598253804459, -291.2158518810209102 ) ) ;
#53787=CARTESIAN_POINT ( 'NONE',  ( -69.34629960582535091, -290.0237909574971695, -203.8479467414003352 ) ) ;
#53789=CARTESIAN_POINT ( 'NONE',  ( -35.11939097372280116, -275.7084878438100759, -343.8206634563861712 ) ) ;
#53790=CARTESIAN_POINT ( 'NONE',  ( 13.17842440672503912, -292.4769948278054699, -324.8244048322745812 ) ) ;
#53792=DIRECTION ( 'NONE',  ( 1.000000000000000000, 0.000000000000000000, 0.000000000000000000 ) ) ;
#53793=CARTESIAN_POINT ( 'NONE',  ( -8.752855232501968175, -290.8993879231106803, -199.6123674590418489 ) ) ;
#53794=CARTESIAN_POINT ( 'NONE',  ( -111.0283494357677085, -286.2166081833692601, -265.4318532408312876 ) ) ;
#53795=CARTESIAN_POINT ( 'NONE',  ( -6.064349368327516032, -286.8865769038594635, -339.6121204724365725 ) ) ;
#53796=CARTESIAN_POINT ( 'NONE',  ( 20.79508455461865424, -288.3470181421716916, -225.2447220087632331 ) ) ;
#53798=CARTESIAN_POINT ( 'NONE',  ( 20.46196134679606971, -287.7246791635639624, -225.5131698956544994 ) ) ;
#53800=CARTESIAN_POINT ( 'NONE',  ( 25.11519868815494050, -294.9632919028105675, -228.1084572948894902 ) ) ;
#53802=CARTESIAN_POINT ( 'NONE',  ( 37.89728070803992921, -288.5763091559493887, -255.9699928602805414 ) ) ;
#53803=CARTESIAN_POINT ( 'NONE',  ( -112.7718771662168535, -276.6884237887530844, -265.9336370287980458 ) ) ;
#53804=CARTESIAN_POINT ( 'NONE',  ( -48.48673000920530285, -277.5234669723861884, -346.5827895998542658 ) ) ;
#53805=CARTESIAN_POINT ( 'NONE',  ( 23.66651032813422972, -291.0289028029738461, -225.7818351594687272 ) ) ;
#53806=CARTESIAN_POINT ( 'NONE',  ( -72.50681190168280921, -279.5997139831050617, -201.8452629067262762 ) ) ;
#53807=CARTESIAN_POINT ( 'NONE',  ( -71.23645610329641897, -299.5823714154043955, -203.8413098687840943 ) ) ;
#53809=CARTESIAN_POINT ( 'NONE',  ( -69.61304295716904278, -283.6272128507254706, -202.6449514173468742 ) ) ;
#53811=CARTESIAN_POINT ( 'NONE',  ( -74.65427059269417498, -275.6939540864842115, -334.5377302799010977 ) ) ;
#53812=CARTESIAN_POINT ( 'NONE',  ( 36.82107716984844359, -279.4041693617803617, -258.8484257117196989 ) ) ;
#53814=CARTESIAN_POINT ( 'NONE',  ( -5.591075499922819603, -275.1219582218917594, -339.7484769946556185 ) ) ;
#53815=CARTESIAN_POINT ( 'NONE',  ( -108.1307173254744072, -298.3406660664528545, -249.8764213167940227 ) ) ;
#53816=CARTESIAN_POINT ( 'NONE',  ( -34.50422900785937941, -281.9376023956479003, -346.9994978463583379 ) ) ;
#53817=CARTESIAN_POINT ( 'NONE',  ( -109.9711776147204034, -297.6220607304188093, -260.5771500789070387 ) ) ;
#53818=CARTESIAN_POINT ( 'NONE',  ( -80.36165112878053662, -298.7981143427669508, -207.0314493906307973 ) ) ;
#53819=CARTESIAN_POINT ( 'NONE',  ( 2.945142243337858456, -274.2758474914076032, -209.3986512255144703 ) ) ;
#53820=CARTESIAN_POINT ( 'NONE',  ( 24.21528019205082316, -294.9707634460075383, -227.4929773961752062 ) ) ;
#53821=CARTESIAN_POINT ( 'NONE',  ( 35.94840406658695997, -288.0157726787018646, -293.9738398002437521 ) ) ;
#53822=CARTESIAN_POINT ( 'NONE',  ( -111.5767603299888435, -276.8124289874544957, -256.2040983486289178 ) ) ;
#53823=CARTESIAN_POINT ( 'NONE',  ( -113.1716504514178752, -290.5527120497221745, -256.9888093382853071 ) ) ;
#53826=CARTESIAN_POINT ( 'NONE',  ( 12.30653773662580619, -287.3995751320486534, -324.2673733040364823 ) ) ;
#53827=CARTESIAN_POINT ( 'NONE',  ( -58.35332334956310518, -289.7803841320211404, -198.3645046191483630 ) ) ;
#53830=CARTESIAN_POINT ( 'NONE',  ( 25.74602580085518966, -287.5663775226341841, -307.3111863164332931 ) ) ;
#53832=CARTESIAN_POINT ( 'NONE',  ( -109.9981041180819687, -285.1802630859983196, -295.1374609723259823 ) ) ;
#53833=CARTESIAN_POINT ( 'NONE',  ( -33.53899619861093129, -291.1576748410219579, -193.6906565508614904 ) ) ;
#53834=CARTESIAN_POINT ( 'NONE',  ( 38.82084841480964599, -283.1824693470330203, -272.7499697835081065 ) ) ;
#53835=CARTESIAN_POINT ( 'NONE',  ( 38.91880072476695318, -282.7901069841477693, -264.2264393889763596 ) ) ;
#53836=CARTESIAN_POINT ( 'NONE',  ( -73.79863336783540717, -283.3836797457146872, -333.6634221105994129 ) ) ;
#53837=CARTESIAN_POINT ( 'NONE',  ( -103.8498035772478119, -297.0582403171705437, -231.4530491659762106 ) ) ;
#53838=CARTESIAN_POINT ( 'NONE',  ( -59.64111142486407857, -275.0725195057470955, -200.2794134251790581 ) ) ;
#53839=CARTESIAN_POINT ( 'NONE',  ( -49.94211009299280590, -289.9108479331492276, -196.7350255217619122 ) ) ;
#53840=CARTESIAN_POINT ( 'NONE',  ( 9.188972840122552554, -297.5684187788447730, -197.0607906701177399 ) ) ;
#53841=ORIENTED_EDGE ( 'NONE', *, *, #87763, .F. ) ;
#53843=CARTESIAN_POINT ( 'NONE',  ( -81.46030306723940839, -285.5772743999670524, -330.3824123368046344 ) ) ;
#53844=CARTESIAN_POINT ( 'NONE',  ( -44.75201475458462852, -296.2233916136306107, -346.7463458733362813 ) ) ;
#53845=CARTESIAN_POINT ( 'NONE',  ( -102.3327996906839275, -285.6578850998902794, -236.8939752081201107 ) ) ;
#53846=CARTESIAN_POINT ( 'NONE',  ( 36.26442877219990635, -274.8856837442878600, -292.2010015832324257 ) ) ;
#53847=CARTESIAN_POINT ( 'NONE',  ( 1.641261442547662597, -293.2100757234092612, -204.0157188802905068 ) ) ;
#53848=CARTESIAN_POINT ( 'NONE',  ( 37.45167714776628287, -285.8494989561767170, -282.7731150850767676 ) ) ;
#53849=CARTESIAN_POINT ( 'NONE',  ( -40.63576438945634806, -292.3450972463186304, -193.4395950645307778 ) ) ;
#53850=CARTESIAN_POINT ( 'NONE',  ( -109.2983355038224005, -291.0530753999199192, -257.6493587272869945 ) ) ;
#53853=CARTESIAN_POINT ( 'NONE',  ( -105.0131974969233823, -260.5199095907283322, -315.5713868923170935 ) ) ;
#53854=CARTESIAN_POINT ( 'NONE',  ( -70.78002839939547641, -287.1391802593108196, -201.7711335959585028 ) ) ;
#53855=CARTESIAN_POINT ( 'NONE',  ( -117.3381139276884966, -270.1608578419545665, -261.3154543817420290 ) ) ;
#53856=CARTESIAN_POINT ( 'NONE',  ( -78.56173964086521266, -282.5421560468634539, -330.9840048780154689 ) ) ;
#53857=CARTESIAN_POINT ( 'NONE',  ( -71.56526471940529177, -277.1586416372951476, -339.3139418428858676 ) ) ;
#53858=CARTESIAN_POINT ( 'NONE',  ( -49.46334835737528834, -281.8974109390292142, -196.5160499806509335 ) ) ;
#53859=CARTESIAN_POINT ( 'NONE',  ( 66.72872018252358828, 46.00066320285807819, -316.9038945764073674 ) ) ;
#53860=CARTESIAN_POINT ( 'NONE',  ( 13.27676825419560203, -280.9355929817181163, -327.6711764478134228 ) ) ;
#53861=CARTESIAN_POINT ( 'NONE',  ( -8.842590557091856596, -284.4469001550755252, -201.3571043685095674 ) ) ;
#53862=CARTESIAN_POINT ( 'NONE',  ( -113.1073802691691839, -274.4481303064853250, -267.5632856924480052 ) ) ;
#53863=CARTESIAN_POINT ( 'NONE',  ( -26.19183625367893598, -295.3987156376396683, -342.5668585929998926 ) ) ;
#53865=CARTESIAN_POINT ( 'NONE',  ( 35.69506761312781151, -292.3499711950225901, -278.9849237609527677 ) ) ;
#53866=CARTESIAN_POINT ( 'NONE',  ( 34.09265066667622790, -276.5668189960217660, -298.9730580085625888 ) ) ;
#53867=CARTESIAN_POINT ( 'NONE',  ( 33.83376145477104302, -275.3375332777842459, -254.0863006109598246 ) ) ;
#53868=CARTESIAN_POINT ( 'NONE',  ( 28.24535536162866833, -273.9504234910574496, -230.5124837694347661 ) ) ;
#53870=CARTESIAN_POINT ( 'NONE',  ( -69.71002884953006173, -271.6259365963096570, -202.6914973942407698 ) ) ;
#53871=CARTESIAN_POINT ( 'NONE',  ( 17.15414218000039526, -295.7190632345941594, -323.9976620302848005 ) ) ;
#53874=CARTESIAN_POINT ( 'NONE',  ( -94.51749362711206004, -284.9859424490852007, -316.2630472235535990 ) ) ;
#53875=CARTESIAN_POINT ( 'NONE',  ( 36.56804806138858766, -283.5365524708048497, -288.0610409790464814 ) ) ;
#53876=CARTESIAN_POINT ( 'NONE',  ( -108.4627552590530968, -284.1240525449600227, -253.4049209915497727 ) ) ;
#53877=CARTESIAN_POINT ( 'NONE',  ( -21.50095326729297085, -275.2456558486217659, -342.4935709810504818 ) ) ;
#53878=CARTESIAN_POINT ( 'NONE',  ( -32.03413807419986625, -284.8448989782980334, -344.4063424466788774 ) ) ;
#53879=CARTESIAN_POINT ( 'NONE',  ( -69.57196504867188480, -275.9641099762362728, -336.6466336187812658 ) ) ;
#53880=CARTESIAN_POINT ( 'NONE',  ( -16.56617244506084674, -275.4065258706298209, -200.0045375989336094 ) ) ;
#53882=CARTESIAN_POINT ( 'NONE',  ( -100.1229642933790984, -279.9424045037632709, -226.0590673475633992 ) ) ;
#53885=CARTESIAN_POINT ( 'NONE',  ( -60.16083807697842190, -287.6200072634221669, -198.0596803194119673 ) ) ;
#53887=CARTESIAN_POINT ( 'NONE',  ( -4.272798959704450894, -293.8018483010718001, -335.6365400018029845 ) ) ;
#53888=CARTESIAN_POINT ( 'NONE',  ( -98.08419835199266856, -289.2701675944013573, -317.5168355214228768 ) ) ;
#53889=CARTESIAN_POINT ( 'NONE',  ( 36.69463280298963070, -285.7652689710423033, -268.3063860241469456 ) ) ;
#53890=CARTESIAN_POINT ( 'NONE',  ( 13.56012671391319024, -285.3563272338353158, -217.1459111527044286 ) ) ;
#53891=CARTESIAN_POINT ( 'NONE',  ( -84.45710032901575914, -289.6329138788665318, -213.2812347063773757 ) ) ;
#53892=CARTESIAN_POINT ( 'NONE',  ( -40.00360392058113490, -287.2230409904963722, -197.0123294858813665 ) ) ;
#53893=CARTESIAN_POINT ( 'NONE',  ( -98.04636780952390041, -275.9518301111650658, -314.4277605498646153 ) ) ;
#53894=CARTESIAN_POINT ( 'NONE',  ( -36.12031628919270787, -287.4369904482509241, -346.5643059251794398 ) ) ;
#53895=CARTESIAN_POINT ( 'NONE',  ( -43.52739389118366375, -287.9742998346473541, -195.5647578969625897 ) ) ;
#53896=CARTESIAN_POINT ( 'NONE',  ( 34.19495515066807201, -285.8492817030654010, -293.4378460432636757 ) ) ;
#53897=CARTESIAN_POINT ( 'NONE',  ( 1.235408126949466112, -283.4648075695793636, -332.6715656782942574 ) ) ;
#53898=CARTESIAN_POINT ( 'NONE',  ( -45.79370798446272062, -291.1590929129508254, -345.1029515984594127 ) ) ;
#53901=CARTESIAN_POINT ( 'NONE',  ( -112.5081904911771318, -298.3741531467688901, -278.0626063502048737 ) ) ;
#53902=CARTESIAN_POINT ( 'NONE',  ( 25.36843145603753769, -278.9957808249042728, -229.1281386727530958 ) ) ;
#53903=CARTESIAN_POINT ( 'NONE',  ( -64.32250657930283921, -290.9061701429879463, -198.3592885442645866 ) ) ;
#53904=CARTESIAN_POINT ( 'NONE',  ( -89.07704497911473140, -294.1939058613223210, -323.0627430589873939 ) ) ;
#53905=CARTESIAN_POINT ( 'NONE',  ( 14.25908599712159486, -280.9936110619752867, -322.7644116494458899 ) ) ;
#53906=CARTESIAN_POINT ( 'NONE',  ( 25.01281134039493637, -273.0795079742320581, -229.7011979500600489 ) ) ;
#53907=CARTESIAN_POINT ( 'NONE',  ( -41.04744583537010527, -296.4149053782379610, -343.7734359737297609 ) ) ;
#53909=CARTESIAN_POINT ( 'NONE',  ( -100.7096567525790078, -271.6948415323470840, -227.5690797961061946 ) ) ;
#53910=CARTESIAN_POINT ( 'NONE',  ( -47.51833934386024794, -293.4196790688521332, -345.6632429621491269 ) ) ;
#53911=CARTESIAN_POINT ( 'NONE',  ( 22.27145705071026782, -294.3783714648906766, -227.1928959682260825 ) ) ;
#53913=CARTESIAN_POINT ( 'NONE',  ( 31.95068112580397468, -294.0418635494150976, -246.7265200021890621 ) ) ;
#53915=CARTESIAN_POINT ( 'NONE',  ( -38.72811899457374807, -281.0895736199433941, -345.7035671683970577 ) ) ;
#53916=CARTESIAN_POINT ( 'NONE',  ( -6.764908165342906621, -294.6392031248318517, -336.6488226740592609 ) ) ;
#53917=CARTESIAN_POINT ( 'NONE',  ( -58.48674883771838751, -283.3180535985534902, -344.4563821424607113 ) ) ;
#53918=CARTESIAN_POINT ( 'NONE',  ( -28.41976538749815973, -282.0845130842482718, -195.2770821648892081 ) ) ;
#53919=CARTESIAN_POINT ( 'NONE',  ( -73.59930161816321004, -285.2514998133198674, -202.3967750621636128 ) ) ;
#53920=CARTESIAN_POINT ( 'NONE',  ( -110.7418340484448862, -288.3635819211841635, -285.0023944294387661 ) ) ;
#53922=CARTESIAN_POINT ( 'NONE',  ( 37.31044519307619822, -279.8318005328021059, -254.4945804494235801 ) ) ;
#53923=CARTESIAN_POINT ( 'NONE',  ( 37.20070123609671242, -286.6994925912204053, -288.4421709853007201 ) ) ;
#53925=CARTESIAN_POINT ( 'NONE',  ( -80.60749199442902579, -297.2501251212485158, -330.1483379166115242 ) ) ;
#53926=CARTESIAN_POINT ( 'NONE',  ( -34.29627077004398927, -278.4398304005497948, -346.7111779306290487 ) ) ;
#53927=CARTESIAN_POINT ( 'NONE',  ( -27.55133941464711711, -279.8465300468889154, -197.9480688981650474 ) ) ;
#53928=CARTESIAN_POINT ( 'NONE',  ( 38.35764393178612153, -293.8959734726582838, -284.5252533351341526 ) ) ;
#53929=CARTESIAN_POINT ( 'NONE',  ( -110.8245891400314207, -282.4070642323220000, -288.0108250370809060 ) ) ;
#53930=CARTESIAN_POINT ( 'NONE',  ( -97.19162719896338842, -279.9340384990928783, -315.5815996233719147 ) ) ;
#53931=CARTESIAN_POINT ( 'NONE',  ( 34.29523675194236176, -292.8117810432837018, -285.6382455006382770 ) ) ;
#53932=CARTESIAN_POINT ( 'NONE',  ( -106.3832319209072210, -270.9413509134250830, -240.5093051803292497 ) ) ;
#53935=CARTESIAN_POINT ( 'NONE',  ( 24.47598140093117891, -293.5984367773336885, -309.3992091009642991 ) ) ;
#53937=CARTESIAN_POINT ( 'NONE',  ( -105.5937364680635966, -287.8380690714489560, -285.9065529553535612 ) ) ;
#53938=CARTESIAN_POINT ( 'NONE',  ( -95.89798262376837101, -272.4216309774337219, -220.5882690116843037 ) ) ;
#53939=CARTESIAN_POINT ( 'NONE',  ( 19.90652774611973541, -288.1746318800582571, -219.5292287197438554 ) ) ;
#53940=CARTESIAN_POINT ( 'NONE',  ( 17.82413554364205410, -288.0675005545263048, -318.2461139030481831 ) ) ;
#53941=CARTESIAN_POINT ( 'NONE',  ( -81.21680477907024454, -279.1809913658900086, -329.5699259632511371 ) ) ;
#53942=CARTESIAN_POINT ( 'NONE',  ( -97.72222600681112681, -298.9017730806181703, -227.5573084651370834 ) ) ;
#53944=CARTESIAN_POINT ( 'NONE',  ( -103.7224464993235244, -277.7693601481302039, -238.9251503143225648 ) ) ;
#53946=CARTESIAN_POINT ( 'NONE',  ( -93.64438738855700706, -296.9353986855291510, -217.7881165983977780 ) ) ;
#53947=CARTESIAN_POINT ( 'NONE',  ( -110.3462528574607262, -292.2832624770505277, -284.9743890083857991 ) ) ;
#53948=CARTESIAN_POINT ( 'NONE',  ( 36.64029018806093063, -294.9215564576508086, -252.1099392021816072 ) ) ;
#53951=CARTESIAN_POINT ( 'NONE',  ( -95.84491834727843695, -290.5889011061078122, -314.2142549186395399 ) ) ;
#53953=CARTESIAN_POINT ( 'NONE',  ( -14.22049088873750478, -290.4883110271226769, -198.1553928893376337 ) ) ;
#53954=CARTESIAN_POINT ( 'NONE',  ( -3.426341716943643867, -298.7991852461717599, -193.3803966899450870 ) ) ;
#53955=CARTESIAN_POINT ( 'NONE',  ( -104.4337324863256526, -272.4496981626587058, -241.3080712163742021 ) ) ;
#53957=CYLINDRICAL_SURFACE ( 'NONE', #55250, 2.395975569037589459 ) ;
#53958=CARTESIAN_POINT ( 'NONE',  ( -112.4474098728420017, -291.9011607344708636, -283.9196297246145946 ) ) ;
#53959=CARTESIAN_POINT ( 'NONE',  ( -19.05039376806008633, -297.3376638359844719, -350.3538533559490702 ) ) ;
#53960=CARTESIAN_POINT ( 'NONE',  ( -46.98576043290659499, -287.9296857604794013, -196.0997641079692642 ) ) ;
#53961=CARTESIAN_POINT ( 'NONE',  ( 6.265240006256610705, -272.6451177045447594, -209.4820650045920445 ) ) ;
#53962=CARTESIAN_POINT ( 'NONE',  ( 31.49732882592432759, -277.0983745798826021, -241.8974049203969514 ) ) ;
#53963=CARTESIAN_POINT ( 'NONE',  ( 0.6648867880497250082, -290.6429958369953397, -206.3547624477920124 ) ) ;
#53964=CARTESIAN_POINT ( 'NONE',  ( -73.48638747381571079, -279.3867989933838203, -336.9631661669442906 ) ) ;
#53966=CARTESIAN_POINT ( 'NONE',  ( 18.56696251739005277, -281.5690458506816185, -317.4774054465676159 ) ) ;
#53967=CARTESIAN_POINT ( 'NONE',  ( -111.5249209800548584, -279.3867733321280298, -289.8637042524648564 ) ) ;
#53968=CARTESIAN_POINT ( 'NONE',  ( 36.60574977127839702, -280.0948240150589186, -250.3167529644021556 ) ) ;
#53969=CARTESIAN_POINT ( 'NONE',  ( -71.72385729004520272, -195.2026553322960751, -357.3366892497529079 ) ) ;
#53970=CARTESIAN_POINT ( 'NONE',  ( 15.85532545509639846, -275.7251389392940837, -215.0176749958938274 ) ) ;
#53972=CARTESIAN_POINT ( 'NONE',  ( -71.11352178364819565, -275.1346028521467701, -201.9347209012333622 ) ) ;
#53973=CARTESIAN_POINT ( 'NONE',  ( -114.2704648735229114, -299.0519495502701943, -270.3937649182068981 ) ) ;
#53977=CARTESIAN_POINT ( 'NONE',  ( -48.09278901894641223, -290.2716825594848729, -342.9288371990923565 ) ) ;
#53978=CARTESIAN_POINT ( 'NONE',  ( -71.43150295606771749, -291.2563136431152770, -338.2717898981143776 ) ) ;
#53979=CARTESIAN_POINT ( 'NONE',  ( -100.3960693493331036, -289.3923899523622936, -307.4478506293191344 ) ) ;
#53980=CARTESIAN_POINT ( 'NONE',  ( -43.65496042878422855, -285.4821942428148986, -193.6288974966489604 ) ) ;
#53982=CARTESIAN_POINT ( 'NONE',  ( 36.22472651994197435, -280.0365765040768906, -276.8414469592522664 ) ) ;
#53983=CARTESIAN_POINT ( 'NONE',  ( 33.44437681840988574, -289.1205248519243582, -247.9535251638666011 ) ) ;
#53984=CARTESIAN_POINT ( 'NONE',  ( -5.753147139932202059, -281.1090146610890770, -336.9548073770945962 ) ) ;
#53985=CARTESIAN_POINT ( 'NONE',  ( -106.7242638539525927, -279.5452974409242870, -294.7496976920084535 ) ) ;
#53986=CARTESIAN_POINT ( 'NONE',  ( 23.10960723032857800, -289.1279196965655842, -317.6946500689371078 ) ) ;
#53987=CARTESIAN_POINT ( 'NONE',  ( -79.09516679938916184, -279.9640859369499708, -210.4058307892098867 ) ) ;
#53988=CARTESIAN_POINT ( 'NONE',  ( -86.24767197844842315, -290.1862100530678958, -211.3328232904735557 ) ) ;
#53989=CARTESIAN_POINT ( 'NONE',  ( -106.5381401926974689, -285.7844977389461292, -236.9543596486820434 ) ) ;
#53990=CARTESIAN_POINT ( 'NONE',  ( 18.30265299723423311, -287.3166245345396987, -217.1501875626344429 ) ) ;
#53991=CARTESIAN_POINT ( 'NONE',  ( -110.2283714244402972, -284.7833906097777685, -265.4673190576978641 ) ) ;
#53992=EDGE_LOOP ( 'NONE', ( #43852, #41746, #82360, #83006, #45421 ) ) ;
#53994=CARTESIAN_POINT ( 'NONE',  ( -66.56131965836367215, -293.5339097416036225, -200.4574748994489539 ) ) ;
#53995=CARTESIAN_POINT ( 'NONE',  ( 20.98078239598116213, -292.9087710980380734, -319.8766337963498358 ) ) ;
#53996=CARTESIAN_POINT ( 'NONE',  ( 34.39262373772408665, -274.8048640757493786, -285.1122273752473575 ) ) ;
#53997=CARTESIAN_POINT ( 'NONE',  ( -113.1049059125042362, -295.7321387567311604, -283.8246259857402265 ) ) ;
#53998=CARTESIAN_POINT ( 'NONE',  ( -101.7200378557766385, -289.5190440767757991, -234.3935975212878873 ) ) ;
#53999=CARTESIAN_POINT ( 'NONE',  ( -73.82110537864811306, -293.7835279315664252, -334.7600854182182957 ) ) ;
#54000=CARTESIAN_POINT ( 'NONE',  ( -60.39818083590582631, -292.9516190491950169, -200.6261575995077919 ) ) ;
#54002=CARTESIAN_POINT ( 'NONE',  ( 7.771451739761555011, -290.6659425388409090, -210.1726681005685862 ) ) ;
#54003=CARTESIAN_POINT ( 'NONE',  ( 34.37138275451705738, -295.2687153460863101, -248.3578371875492223 ) ) ;
#54004=CARTESIAN_POINT ( 'NONE',  ( 33.93283969678166301, -288.7147595850378252, -287.1940743976730914 ) ) ;
#54007=CARTESIAN_POINT ( 'NONE',  ( -28.76270564614470970, -278.9239159720255543, -345.2788136133865464 ) ) ;
#54008=CARTESIAN_POINT ( 'NONE',  ( -95.85586566241099149, -276.6773954718863138, -319.8192204087628738 ) ) ;
#54009=CARTESIAN_POINT ( 'NONE',  ( -30.49217837075662629, -297.3330341154982648, -193.5234988838759875 ) ) ;
#54010=CARTESIAN_POINT ( 'NONE',  ( -75.21782698397862532, -277.6234137888233704, -206.2182377461876115 ) ) ;
#54011=CARTESIAN_POINT ( 'NONE',  ( -82.09308442490045366, -276.0510868019468376, -332.0356995951354406 ) ) ;
#54012=CARTESIAN_POINT ( 'NONE',  ( -103.2175812133921795, -294.7969091626975455, -303.0585572695978840 ) ) ;
#54014=CARTESIAN_POINT ( 'NONE',  ( -44.59524583593257319, -298.7609995928901867, -197.5096093526454126 ) ) ;
#54016=CARTESIAN_POINT ( 'NONE',  ( -43.08268294367599793, -287.1444101556076021, -345.4973137837422996 ) ) ;
#54017=CARTESIAN_POINT ( 'NONE',  ( -2.911783122493571963, -274.3539869446985335, -205.9904661332122089 ) ) ;
#54018=CARTESIAN_POINT ( 'NONE',  ( 28.90374401279980532, -288.0635153542899047, -309.6108457596720314 ) ) ;
#54019=CARTESIAN_POINT ( 'NONE',  ( -102.6495905338611152, -275.0486224168494687, -233.0422515417800753 ) ) ;
#54020=CARTESIAN_POINT ( 'NONE',  ( -111.6275497342932965, -294.4303608835563182, -279.8127487419566819 ) ) ;
#54021=CARTESIAN_POINT ( 'NONE',  ( -71.67578070230914022, -282.6914594827607630, -339.1021518149162262 ) ) ;
#54023=CARTESIAN_POINT ( 'NONE',  ( -108.6974721796673009, -276.8521163581933138, -247.1011516359438929 ) ) ;
#54025=CARTESIAN_POINT ( 'NONE',  ( -110.1854662083769796, -289.2290494336387496, -279.3564638845061836 ) ) ;
#54028=CARTESIAN_POINT ( 'NONE',  ( -108.9024742553985874, -288.8421187518065381, -247.8667052473525132 ) ) ;
#54029=CARTESIAN_POINT ( 'NONE',  ( 9.914998316094164821, -276.2366864732580325, -213.7477589742381383 ) ) ;
#54030=CARTESIAN_POINT ( 'NONE',  ( 39.03144406008818379, -283.0076414011805355, -272.7588540303314062 ) ) ;
#54031=CARTESIAN_POINT ( 'NONE',  ( -35.49620289696337494, -296.0952583471702724, -195.0065285614429911 ) ) ;
#54032=CARTESIAN_POINT ( 'NONE',  ( -61.53472301329966854, -283.3752504545788042, -339.2888606260656843 ) ) ;
#54033=CARTESIAN_POINT ( 'NONE',  ( -57.03663203377729474, -275.2185029534903720, -199.4032152805806390 ) ) ;
#54034=CARTESIAN_POINT ( 'NONE',  ( 34.05308873701784478, -276.5660847958113777, -286.3989159558601045 ) ) ;
#54035=CARTESIAN_POINT ( 'NONE',  ( -19.37223705524605677, -284.8212877209050475, -343.2301662594349523 ) ) ;
#54036=ORIENTED_EDGE ( 'NONE', *, *, #45976, .F. ) ;
#54038=CARTESIAN_POINT ( 'NONE',  ( 24.88502695502878836, -293.9876565002855955, -315.7356637823843357 ) ) ;
#54039=CARTESIAN_POINT ( 'NONE',  ( -104.4813085449890622, -286.0987512858225159, -303.1005911705772178 ) ) ;
#54041=CARTESIAN_POINT ( 'NONE',  ( -111.2869819898779866, -281.6237833571633473, -305.9350535429201159 ) ) ;
#54042=CARTESIAN_POINT ( 'NONE',  ( -37.13768075069169328, -276.2467958809954780, -347.2124025583008233 ) ) ;
#54043=CARTESIAN_POINT ( 'NONE',  ( -113.4532250340788693, -288.9056318710334494, -274.0321110462006118 ) ) ;
#54044=CARTESIAN_POINT ( 'NONE',  ( -5.718016765509383426, -284.1487660287102130, -336.9381312271985394 ) ) ;
#54045=CARTESIAN_POINT ( 'NONE',  ( -85.75133073334696121, -279.4928756592313448, -326.4154309696538121 ) ) ;
#54046=CARTESIAN_POINT ( 'NONE',  ( 7.185722172988596057, -288.0705758170323065, -208.1999471684363527 ) ) ;
#54047=CARTESIAN_POINT ( 'NONE',  ( -16.38666980254915728, -282.3231646714657472, -198.3480125763209969 ) ) ;
#54048=CARTESIAN_POINT ( 'NONE',  ( 38.72727800654578800, -275.5684704136840537, -258.3383640673652621 ) ) ;
#54049=CARTESIAN_POINT ( 'NONE',  ( -77.81670765481877083, -277.4128324662781893, -335.9270777748633350 ) ) ;
#54050=CARTESIAN_POINT ( 'NONE',  ( -98.07140855564131243, -299.0617600786443404, -227.3121143527116317 ) ) ;
#54052=CARTESIAN_POINT ( 'NONE',  ( 21.27581636871892101, -283.4090924074130839, -223.5744983911110353 ) ) ;
#54053=CARTESIAN_POINT ( 'NONE',  ( -75.14274473285500733, -295.6940649792166482, -204.6397676035028894 ) ) ;
#54055=CARTESIAN_POINT ( 'NONE',  ( -51.29877536669942373, -276.7430977463810677, -342.0771447286907119 ) ) ;
#54056=CARTESIAN_POINT ( 'NONE',  ( 23.30900661503532589, -276.1292450733118926, -223.5476736826244064 ) ) ;
#54057=CARTESIAN_POINT ( 'NONE',  ( -24.99453589156636824, -287.9717748042413632, -197.3329386761267870 ) ) ;
#54058=CARTESIAN_POINT ( 'NONE',  ( -112.7078449822472521, -298.2240461152812259, -258.3345120083503730 ) ) ;
#54059=CARTESIAN_POINT ( 'NONE',  ( -81.62956339276007611, -296.8449640314987619, -332.9286472458695130 ) ) ;
#54060=CARTESIAN_POINT ( 'NONE',  ( -34.82039927017625303, -294.0840653045207773, -195.5702664614639730 ) ) ;
#54061=CARTESIAN_POINT ( 'NONE',  ( -93.56953765346997898, -277.2397834047061451, -220.9608803310800340 ) ) ;
#54062=CARTESIAN_POINT ( 'NONE',  ( -35.65419579538057349, -281.9936081159942773, -195.9275958805040432 ) ) ;
#54063=CARTESIAN_POINT ( 'NONE',  ( -87.04394116810205162, -295.4334165023100809, -214.9445010610481859 ) ) ;
#54064=CARTESIAN_POINT ( 'NONE',  ( -87.48600437731853674, -285.6030721609664056, -327.2277537317200427 ) ) ;
#54066=CARTESIAN_POINT ( 'NONE',  ( 32.57251878286696467, -286.1809118724847849, -248.2684866787102180 ) ) ;
#54067=CARTESIAN_POINT ( 'NONE',  ( -97.80750439109840499, -248.8887263784241668, -333.8114341845347326 ) ) ;
#54069=CARTESIAN_POINT ( 'NONE',  ( 33.73187304974455714, -286.9972326927515951, -253.5549114796776848 ) ) ;
#54071=CARTESIAN_POINT ( 'NONE',  ( -90.21503184404798503, -284.8582719452872425, -325.9848275579730057 ) ) ;
#54072=CARTESIAN_POINT ( 'NONE',  ( -2.907435594079280428, -274.8538673597004163, -205.9688132184403457 ) ) ;
#54073=CARTESIAN_POINT ( 'NONE',  ( -23.84072744710957537, -285.0157497171977639, -194.9033828854142030 ) ) ;
#54074=CARTESIAN_POINT ( 'NONE',  ( -11.24545392176759862, -291.3045843531622268, -198.1909580222750265 ) ) ;
#54075=CARTESIAN_POINT ( 'NONE',  ( 39.38500731920789377, -282.5236990018889855, -272.7761907766800391 ) ) ;
#54076=CARTESIAN_POINT ( 'NONE',  ( -107.8791836013111549, -280.4455523805548296, -241.2549128642503149 ) ) ;
#54077=CARTESIAN_POINT ( 'NONE',  ( 36.15425854676276174, -281.5977567520299658, -247.4681419858337676 ) ) ;
#54078=CARTESIAN_POINT ( 'NONE',  ( 17.36665895637873192, -285.6952119285918457, -314.0302885647153062 ) ) ;
#54079=CARTESIAN_POINT ( 'NONE',  ( -89.67988014755925974, -230.8544109942510545, -347.9892254545792412 ) ) ;
#54080=ORIENTED_EDGE ( 'NONE', *, *, #73503, .T. ) ;
#54081=CARTESIAN_POINT ( 'NONE',  ( -15.83008848003553481, -278.7735471720542364, -342.0902782102641595 ) ) ;
#54082=CARTESIAN_POINT ( 'NONE',  ( 44.27645291422682305, 12.81384402874245332, -331.5602518763756734 ) ) ;
#54083=CARTESIAN_POINT ( 'NONE',  ( 36.09929062543904621, -279.7454315888630845, -283.7843006428992112 ) ) ;
#54084=CARTESIAN_POINT ( 'NONE',  ( -6.192328742830734534, -296.4085921700738595, -339.6697803456366955 ) ) ;
#54085=CARTESIAN_POINT ( 'NONE',  ( -98.82352221797420100, -295.3531143395752565, -309.9997652490462201 ) ) ;
#54086=CARTESIAN_POINT ( 'NONE',  ( -61.66317845459105484, -291.2521894909195339, -197.3119079829695295 ) ) ;
#54088=CARTESIAN_POINT ( 'NONE',  ( -105.9760417171177096, -295.5614950743363920, -236.7763975591273606 ) ) ;
#54089=CARTESIAN_POINT ( 'NONE',  ( -5.465133247984220510, -287.0254846115550436, -336.9218038393461825 ) ) ;
#54090=CARTESIAN_POINT ( 'NONE',  ( 36.94415581737101206, -295.4175296656277396, -270.7430259030278421 ) ) ;
#54091=CARTESIAN_POINT ( 'NONE',  ( 30.40993689606916206, -288.4862012691365294, -241.7520533262001550 ) ) ;
#54093=CARTESIAN_POINT ( 'NONE',  ( 33.20508585027005921, -294.8815766906969316, -300.7604272105157861 ) ) ;
#54094=CARTESIAN_POINT ( 'NONE',  ( -95.16129769550697404, -284.4159489726229140, -315.0456464905165035 ) ) ;
#54095=CARTESIAN_POINT ( 'NONE',  ( -105.6108339533654998, -294.8960019698889141, -305.2247252189152391 ) ) ;
#54096=CARTESIAN_POINT ( 'NONE',  ( -113.5074846170469698, -291.4870196487693761, -259.8256539460477370 ) ) ;
#54097=CARTESIAN_POINT ( 'NONE',  ( -112.2587832337740963, -291.2637922075107326, -252.8409135743088143 ) ) ;
#54098=CARTESIAN_POINT ( 'NONE',  ( -71.17087407533799137, -289.6784229638754482, -335.0636241075252428 ) ) ;
#54101=CARTESIAN_POINT ( 'NONE',  ( -100.5327758358061772, -298.9715923473462453, -228.5380401843699758 ) ) ;
#54102=CARTESIAN_POINT ( 'NONE',  ( -35.51777851591091917, -272.8694600128239358, -193.7668436873507574 ) ) ;
#54103=CARTESIAN_POINT ( 'NONE',  ( 10.05186962290427921, -281.4390921062220059, -326.2602082448455576 ) ) ;
#54106=CARTESIAN_POINT ( 'NONE',  ( 39.64574763058467255, -275.0700209352943375, -271.1772532756260148 ) ) ;
#54107=CARTESIAN_POINT ( 'NONE',  ( -108.9775298495964506, -294.8053684692861225, -287.7064578780840520 ) ) ;
#54108=CARTESIAN_POINT ( 'NONE',  ( 14.61244068419422426, -278.1722401832040532, -323.4575643368825695 ) ) ;
#54109=CARTESIAN_POINT ( 'NONE',  ( 0.09679817608398202933, -272.6957045914627429, -206.2430459753439322 ) ) ;
#54110=CARTESIAN_POINT ( 'NONE',  ( -108.3498474304395245, -297.5127431717701256, -288.9842317282793829 ) ) ;
#54111=CARTESIAN_POINT ( 'NONE',  ( -110.6932029985250523, -297.6171126579783959, -271.4815037568844787 ) ) ;
#54113=CARTESIAN_POINT ( 'NONE',  ( -111.8229346153797223, -298.3563747867192433, -254.2070924821041444 ) ) ;
#54114=CARTESIAN_POINT ( 'NONE',  ( -101.3092036791678794, -271.1047608426662237, -230.5294058557962842 ) ) ;
#54115=CARTESIAN_POINT ( 'NONE',  ( 18.91684969054837495, -294.8646757181084013, -317.0394667196880505 ) ) ;
#54116=CARTESIAN_POINT ( 'NONE',  ( -65.53606030848951036, -290.2508619757775818, -202.3735825817680336 ) ) ;
#54118=CARTESIAN_POINT ( 'NONE',  ( 26.87574231574916439, -275.4868107776628676, -227.9860428891059883 ) ) ;
#54120=CARTESIAN_POINT ( 'NONE',  ( -104.3805482693073543, -273.1086193435667155, -241.3402251240709688 ) ) ;
#54122=CARTESIAN_POINT ( 'NONE',  ( -31.73300502818941027, -284.9616076511811116, -345.5202890343200579 ) ) ;
#54123=CARTESIAN_POINT ( 'NONE',  ( -63.75755852931569478, -282.0743193041981272, -342.1629334006395311 ) ) ;
#54125=CARTESIAN_POINT ( 'NONE',  ( -101.9185556427580224, -283.2804724647268699, -304.8554705005352616 ) ) ;
#54126=CARTESIAN_POINT ( 'NONE',  ( -49.81497601744149506, -281.2106031423585932, -344.5382415850646112 ) ) ;
#54127=CARTESIAN_POINT ( 'NONE',  ( 36.17667299571633066, -274.0714121579113680, -266.1229832589045827 ) ) ;
#54128=CARTESIAN_POINT ( 'NONE',  ( 4.212006058458619862, -282.6119890591320996, -207.8635962137862236 ) ) ;
#54132=CARTESIAN_POINT ( 'NONE',  ( -65.90820487019962570, -272.0844762455563455, -199.7043674272825342 ) ) ;
#54133=CARTESIAN_POINT ( 'NONE',  ( -76.82958269729145684, -279.5793236916941851, -334.3804507435912683 ) ) ;
#54136=CARTESIAN_POINT ( 'NONE',  ( -105.6924460988564931, -286.0518421878123831, -302.5712052283816433 ) ) ;
#54139=CARTESIAN_POINT ( 'NONE',  ( -21.61033311015171066, -286.8504457223311306, -343.7452474685937887 ) ) ;
#54141=CARTESIAN_POINT ( 'NONE',  ( -93.90982623053319855, -296.0066882905446164, -223.5742998329805573 ) ) ;
#54142=CARTESIAN_POINT ( 'NONE',  ( -83.32970995497004196, -287.8296703210663736, -328.6360562458374375 ) ) ;
#54143=CARTESIAN_POINT ( 'NONE',  ( 180.5468918863934960, 256.3577768311903355, -167.2605672291198857 ) ) ;
#54144=CARTESIAN_POINT ( 'NONE',  ( -107.8765914782961630, -294.2197028893193078, -296.0057290955219287 ) ) ;
#54145=CARTESIAN_POINT ( 'NONE',  ( 21.56737458551660680, -285.3744988849808237, -221.8592760431354236 ) ) ;
#54146=CARTESIAN_POINT ( 'NONE',  ( 34.22644608494959328, -282.9165391619682168, -252.2975909449990297 ) ) ;
#54147=CARTESIAN_POINT ( 'NONE',  ( 8.578378750397638086, -280.6725419322424955, -330.9030073413592277 ) ) ;
#54148=CARTESIAN_POINT ( 'NONE',  ( -21.12933984521924557, -288.8382949273853910, -341.5380761506264662 ) ) ;
#54149=CARTESIAN_POINT ( 'NONE',  ( -67.56474743446976561, -281.0729772658729644, -203.2508849506107538 ) ) ;
#54150=CARTESIAN_POINT ( 'NONE',  ( -43.77545601388165153, -280.7717445389827162, -197.4327343074002954 ) ) ;
#54151=CARTESIAN_POINT ( 'NONE',  ( 24.51627414453345466, -290.1141541016406222, -313.4855948307017002 ) ) ;
#54152=CARTESIAN_POINT ( 'NONE',  ( -74.60450101871616368, -295.7001477204482853, -337.8039411495329318 ) ) ;
#54154=CARTESIAN_POINT ( 'NONE',  ( -108.0775012092738905, -272.9411894920630175, -239.8051244167468781 ) ) ;
#54155=CARTESIAN_POINT ( 'NONE',  ( -38.95791226330022283, -294.0116653546011776, -195.7338128963984332 ) ) ;
#54157=CARTESIAN_POINT ( 'NONE',  ( 21.27581636871892101, -277.4090924074130839, -223.5744983911110353 ) ) ;
#54159=CARTESIAN_POINT ( 'NONE',  ( 36.69098792003511988, -273.3844072212879723, -257.2801438398193454 ) ) ;
#54161=CARTESIAN_POINT ( 'NONE',  ( -113.4362467417314377, -294.8900214476975066, -275.2673441416986861 ) ) ;
#54162=CARTESIAN_POINT ( 'NONE',  ( 9.556821120296728367, -274.0655007057300168, -214.2196831090664659 ) ) ;
#54163=CARTESIAN_POINT ( 'NONE',  ( -110.8122372985201594, -291.9893335689440619, -276.7087138429859010 ) ) ;
#54164=B_SPLINE_SURFACE_WITH_KNOTS ( 'NONE', 3, 3, ( 
 ( #68811, #84854, #70683, #54578, #18604, #47469, #18371, #19773, #41534, #77544, #47712, #56240, #83693, #55309, #76141, #25932, #4633, #48643, #11275, #54815, #20252, #70460, #42000, #18854, #76612, #33507, #70914, #12204, #11735, #78024, #13164, #92664, #33047, #62413, #34919, #49128, #40128, #40588, #84162, #69045, #54352, #5587, #69975, #19310, #34459, #63367, #4174, #90773, #41048, #91255, #61937, #6047, #69502, #26419, #92197, #63832, #48172, #83226, #12694, #85102, #77073, #5115, #33993, #62896, #91732, #26885, #55772, #84625, #27353, #21175, #72764, #36776, #57638, #7886, #22561, #66145, #79423, #43415, #27836, #86026, #29217, #35855, #50983, #79868, #71384, #56725, #15008, #80324, #87414, #15464, #78940, #78484, #85571, #65227, #42473, #71861, #50044, #51435, #20718, #42955, #13620, #43867, #86961, #49588, #72310, #810, #86482, #6517, #35395, #28755, #14090, #64315, #93140, #6982, #21647, #93597, #332, #64772, #50525, #65696, #7431, #58116, #28295, #29690, #58574, #57185, #14558, #36311, #44336, #22114, #73247, #8358, #37241, #67532, #82649, #39532, #74152, #8809, #9755, #38147, #67063, #87874, #60890, #38629, #75553, #23956, #89269, #30143, #59971, #46192, #31083, #52831, #89740, #16396, #31541, #2662, #88809, #15943, #9269, #60429, #59027, #75097, #24419, #81709, #66596, #23024, #37690, #2199, #45247, #45714, #73700, #16858, #59504, #53300, #82185, #10677, #24902, #74626, #53782, #1717, #17341, #30601, #46651, #10206, #3114, #81249, #51902, #39075, #67988, #88355, #31997, #17798, #1261, #80795, #23506, #44797, #52374, #4515, #48526, #63253, #13056, #26298, #84050, #68454, #32931, #69856, #76496, #91618, #26773, #18258, #3588, #55658, #27239, #34346, #56127, #25816, #25357, #32478, #12088, #83106, #18732, #61823, #92084, #61375, #83571, #54237, #84511, #33876, #90208, #19196, #41417, #33392, #47111, #76019, #69383, #90655, #11151, #40013, #54696, #62291, #40465, #40936, #47593, #91128, #77427, #48056, #4991, #68930, #19657, #5476, #4061, #55192, #11620, #12567, #62785, #76960, #70350, #84980, #20132, #49016, #77914, #5938, #70803, #34810, #63723, #92548, #41892, #6163, #77663, #20832, #63012, #34572, #69151, #5239, #85222, #70098, #91843, #35033, #55419, #70572, #12815, #34110, #54931, #19423, #41655, #4279, #20373, #5697, #26998, #11845, #33157, #47817, #41161, #84272, #84739, #18964, #48285, #4743, #63481, #27466, #49701, #63947, #19887, #92786, #40695, #55886, #69614, #56358, #85685, #33623, #92311, #42114, #26531, #62048, #77188, #48758, #62532, #49244, #71030, #27954, #78139, #91373, #13277, #56844, #78597, #40236, #90882, #26045, #83811, #76719, #12317, #71980, #15121, #21774, #36898, #65814, #57302, #13739, #924, #66258, #73359, #1373, #64890, #64431, #52027, #51097, #28411, #57758, #7099, #37351, #71504, #28870, #93257, #29804, #72881, #6637, #58234, #80437, #72430, #42589, #35517, #14677, #35970, #86144, #21294, #82458, #43533, #79538, #79984, #86604, #7547, #22676, #87078, #43983, #50167, #58685, #44453, #79064, #36431, #50650, #51548, #8006, #14216, #43076, #65347, #15582, #30255, #454, #29341, #22227, #8471, #59146, #87991, #23144, #46766, #24539, #61487, #9868, #75211, #16057, #45843, #32121, #16978, #38743, #75667, #2321, #17457, #53423, #74748, #1839, #60087, #82307, #44910, #61017, #46307, #67648, #52488, #73813, #88474, #81827, #31202, #31655, #59627, #88926, #45364, #10326, #68105, #90319, #10791, #60546, #39652, #81363, #2774, #16513, #3230, #32597, #74267, #25473, #37804, #8926, #89384, #39193, #17915, #89863, #25023, #66710, #53895, #68575, #30726, #24074, #3712, #80912, #82763, #23621, #9390, #38274, #67187, #52950, #58376, #66852, #609, #65956, #86757, #36577, #15268, #30402, #29016, #65491, #30879, #52173, #52626, #29493, #87219, #44127, #81506, #22827, #22366, #88614, #23760, #9539, #43674, #73032, #45507, #59772, #21919, #51240, #1067, #57903, #65033, #81054, #80584, #29946, #16199, #73950, #50793, #7691, #51696, #8159, #14819, #16653, #80128, #79677, #66400, #72570, #37044, #58831, #1516, #87676, #15738, #74409, #134, #59294, #44599, #73504, #8614, #37490, #88141, #23298, #45049, #9065, #37943, #1987, #60228, #10469, #18515, #46911, #38880, #10936, #74898, #54971, #46452, #61624, #25161, #11418, #24695, #81971, #90917, #39803, #67334, #47853, #82903, #45993, #68725, #2465, #67788, #39334, #47380, #76756, #68253, #75811, #54035, #32735, #19000, #4315, #3376, #83848, #83366, #2913, #38424, #33193, #90456, #24217, #31342, #17601, #69186, #18058, #82453, #31798, #62084, #89068, #53578, #53092, #25614, #3855, #17127, #54496, #40270, #32264, #10010, #60691, #61170, #89531, #75353, #90006, #76293, #26083, #77702, #78175, #63048, #41689, #20868, #56400, #49279, #62570, #92827, #42626, #48322, #70606, #70138, #56882, #13312, #40733, #19456, #33660, #42151, #93297, #50203, #84773, #77223, #20410, #48793, #12851, #4779, #71545, #71069, #86182, #34608, #6201, #69650, #5734, #85722, #63519, #92346, #6679, #27032, #35067, #63987, #27501, #26566, #19922, #27990, #91411, #49738, #78637, #85261, #12351, #55454, #41201, #13777, #55921, #35556, #84305, #64469, #5275, #28447, #57341, #21334, #11882, #34143, #91878, #50687, #80023, #79573, #1409, #30768, #14716, #59668, #73398, #80950, #65383, #72020, #497, #36941, #43569, #58724, #16096, #44947, #59184, #72466, #30296, #88028, #15164, #23186, #73847, #23658, #65854, #962, #79107, #7583, #80473, #87115, #8508, #37387, #28908, #14256, #66297, #37842, #8963, #66748, #36469, #36010, #43114, #22713, #29, #57796, #29380, #58274, #15623, #52068, #88511, #1874, #87568, #7137, #22265, #44022, #51140, #64927, #86646, #72920, #21812, #8047, #29841, #51588, #44494, #45883, #24576, #24110, #46346, #75704, #10828, #82799, #52991, #53930, #17950, #31693, #46801, #68614, #54386, #53465, #82345, #52525, #81865, #68146, #67684, #61058, #89900, #67230, #81400, #39688, #61521, #3749, #90352, #74790, #38315, #16548, #3266, #31238, #2811, #9907, #25509, #74303, #38780, #2360, #32631, #25058, #9427, #10362, #45404, #32156, #60124, #88964, #17014, #60587, #75247, #89422, #17493, #39227, #15451, #15931, #797, #73234, #52361, #87861, #80782, #319, #30587, #74138, #79855, #8345, #7872, #88342, #44785, #72296, #50971, #65215, #73686, #31070, #81696, #22548, #14994, #51889, #80312, #44322, #36298, #9256, #8796, #23944, #66133, #37675, #7416, #37228, #23493, #1248, #30130, #38133, #58560, #66584, #1704, #59014, #58103, #51422, #59489, #29203, #81236, #16383, #23010, #43853, #86949, #72751, #45233, #87401, #67048, #2185, #59958, #88797, #29677, #52816, #43401, #22102, #36762, #65683, #4051, #47583, #53286, #75540, #75084, #61811, #18249, #45700, #24407, #38616, #83094, #4503, #55182, #89726, #82172, #25345, #53770, #82636, #9741, #76487, #54226, #91116, #39520, #11139, #74612, #10665, #90644, #46639, #68441, #11610, #31985, #47101, #76008, #3574, #31529, #24890, #40002, #67520, #25806, #68919, #32464, #17329, #2650, #46179, #17786, #60878, #61363, #89256, #90197, #10194, #32921, #54686, #26286, #40455, #83560, #69373, #39063, #18720, #67976, #33382, #62281, #3102, #16844, #60416, #85909, #70341, #76951, #5467, #41883, #19648, #63714, #21061, #49928, #64193, #77417, #35265, #93025, #20120, #28182 ),
 ( #34337, #40926, #13505, #49475, #48046, #34799, #57071, #49005, #28639, #84041, #84971, #48517, #4980, #19186, #41406, #77903, #12556, #78825, #85458, #12078, #91609, #69847, #56604, #71744, #33866, #63244, #26764, #92539, #27229, #56118, #62776, #13970, #27706, #64658, #13046, #78366, #55649, #70794, #42828, #5929, #20605, #6872, #92075, #42353, #71266, #6394, #84502, #35744, #93486, #86373, #37577, #1150, #80215, #29099, #50402, #65116, #58459, #72653, #8248, #36197, #7775, #22005, #87760, #44687, #66940, #52260, #37130, #81140, #57992, #87303, #86846, #73588, #9153, #50875, #38032, #51784, #59383, #43754, #79308, #36660, #15354, #79757, #66037, #88234, #23392, #66488, #14898, #8697, #1604, #22450, #30488, #16284, #2079, #44214, #73121, #57528, #65580, #58914, #695, #80673, #15829, #7319, #21524, #45135, #74036, #14449, #43306, #29579, #72201, #219, #30032, #51322, #22914, #24306, #55890, #88699, #46080, #81594, #55423, #91377, #23847, #76723, #5243, #90886, #70576, #30969, #31887, #89157, #45599, #59858, #82063, #60778, #3001, #4747, #17219, #26049, #41165, #11849, #69619, #16743, #19427, #63016, #67423, #27002, #2551, #54935, #31430, #48289, #77667, #60319, #12819, #26535, #34114, #74988, #52713, #10099, #83815, #53184, #40699, #91847, #84744, #12321, #38966, #77192, #70102, #18968, #19891, #48762, #74500, #47821, #33627, #9631, #67878, #62536, #84276, #41659, #38518, #49248, #5701, #86608, #58238, #65351, #87082, #56848, #56363, #43988, #43080, #20377, #49705, #92790, #29345, #63485, #20836, #85226, #28875, #64894, #92316, #50171, #72434, #64435, #34576, #27470, #6641, #63951, #78143, #13281, #85689, #35521, #71508, #71985, #78601, #93261, #14681, #79068, #7103, #42118, #21778, #36436, #71034, #28415, #27958, #50654, #35974, #6168, #35037, #13744, #21998, #22231, #42593, #57306, #86148, #14220, #21299, #57762, #79542, #458, #43537, #79988, #7551, #51101, #15125, #37807, #24077, #8929, #30729, #67651, #87994, #9393, #45367, #66714, #87531, #52030, #74270, #8010, #52953, #16516, #1842, #44456, #65819, #80440, #73816, #23147, #23624, #51552, #80915, #37354, #38277, #60090, #82310, #2777, #52491, #45846, #59630, #17460, #72885, #88477, #66261, #22679, #36902, #30258, #81366, #44913, #67190, #59150, #2325, #81831, #31205, #88929, #29807, #16981, #9871, #15585, #74751, #1376, #38747, #31658, #927, #73362, #58688, #60549, #89388, #8474, #16060, #24542, #53426, #83229, #18375, #39196, #12207, #83696, #26888, #69048, #40591, #75215, #11278, #91258, #76144, #4177, #41052, #61490, #76615, #18857, #40131, #61020, #25476, #47715, #10329, #26422, #11738, #33050, #17919, #68108, #53898, #47233, #90322, #90777, #25026, #54356, #10795, #69505, #33510, #55775, #69978, #25936, #5119, #46769, #61940, #75670, #62416, #91735, #39655, #84628, #4636, #48175, #32600, #3233, #54818, #55313, #68579, #84165, #77076, #33996, #19313, #3715, #62899, #46310, #32124, #89866, #82766, #58118, #71388, #35398, #19776, #78027, #21178, #27839, #42958, #71864, #63370, #48647, #6985, #72313, #14561, #7434, #70917, #70463, #77547, #86029, #34462, #63836, #13167, #43418, #12698, #34922, #5590, #35858, #78944, #41538, #64318, #36315, #92200, #92667, #27356, #64775, #14094, #56244, #93143, #86486, #78487, #85105, #20255, #20721, #42003, #49131, #6050, #56728, #49591, #85574, #50047, #13623, #42476, #28758, #28298, #93600, #6520, #57641, #50528, #21651, #65230, #335, #29220, #88357, #22116, #812, #15010, #59507, #74629, #31543, #66146, #29692, #1719, #30145, #59028, #79870, #52835, #30604, #67535, #15945, #81251, #50985, #51905, #38151, #23026, #44798, #81711, #8360, #23507, #52376, #80797, #7889, #1263, #16398, #43869, #67067, #45249, #73702, #58576, #72766, #87416, #87875, #37243, #37691, #65698, #8811, #51437, #74154, #9270, #2664, #16861, #66597, #45718, #22563, #2202, #80326, #31086, #38632, #15467, #86963, #59974, #88812, #73249, #36779, #23959, #9757, #44339, #40016, #91132, #26302, #40469, #53784, #11623, #69386, #90211, #4519, #55195, #4995, #18261, #76023, #60433, #24905, #61826, #68458, #83574, #18736, #10208, #89271, #47597, #19199, #84052, #48059, #17800, #17343, #24421, #4064, #75099, #10679, #82651, #61378, #82189, #31999, #39535, #25819, #53302, #60894, #76963, #76499, #12092, #46653, #89744, #3592, #40939, #47114, #75557, #69859, #46194, #39077, #67991, #32481, #3117, #25360, #54240, #83110, #11155, #68933, #32934, #33395, #90659, #54699, #62294, #42841, #26776, #70353, #20616, #13059, #77430, #79321, #56130, #48529, #35278, #19661, #63256, #84983, #64206, #63726, #92087, #93496, #28649, #93036, #27720, #50416, #34349, #27243, #42365, #12572, #34813, #20136, #28192, #71277, #55662, #5941, #13981, #6404, #49020, #57081, #5479, #14459, #41895, #85920, #49486, #6882, #77917, #41421, #86383, #21071, #62788, #43316, #78376, #70807, #49941, #91621, #92551, #56618, #71757, #72212, #85469, #78835, #13515, #35755, #33880, #57540, #64668, #84514, #21534, #36670, #23857, #66951, #59393, #86860, #229, #80226, #38043, #51793, #58005, #65127, #80684, #1159, #2091, #22923, #88246, #29109, #15839, #30981, #22015, #15362, #59869, #52723, #30042, #87772, #50885, #66497, #23404, #30499, #705, #9165, #65592, #45609, #44696, #79766, #51332, #29589, #88709, #14908, #22459, #43764, #52271, #1615, #72665, #73597, #74046, #66047, #7328, #36208, #8258, #58468, #7784, #87312, #44223, #37139, #73132, #8708, #58923, #37586, #16294, #81150, #45147, #81606, #16755, #11517, #17229, #39434, #38976, #25710, #75912, #9643, #82072, #2560, #47009, #62185, #19098, #53681, #46091, #83003, #17698, #46550, #67433, #40364, #18155, #55077, #3478, #68827, #38530, #68350, #54593, #10569, #32370, #69281, #89627, #11037, #39906, #61270, #89166, #82548, #3956, #31439, #83464, #32829, #90105, #74997, #60329, #10109, #75451, #24796, #25256, #53194, #54133, #67888, #61719, #90551, #83946, #4410, #18620, #33289, #3011, #47485, #31897, #76394, #26185, #60789, #74511, #91017, #24317, #34240, #40828, #63146, #5830, #77322, #27604, #78726, #13869, #28086, #41303, #92924, #56973, #77800, #85811, #42721, #86271, #34703, #63616, #47951, #12455, #49377, #56013, #71166, #6294, #91509, #76854, #35163, #6770, #71638, #35645, #5373, #4879, #70240, #91977, #27130, #64562, #92441, #19552, #93386, #28539, #11980, #26665, #84870, #57430, #69748, #33763, #20020, #48898, #62675, #55555, #64085, #56501, #12950, #20962, #49829, #84403, #48418, #85360, #41788, #70699, #20509, #78270, #13409, #42252, #7223, #50775, #72552, #22808, #51221, #79660, #81036, #16180, #80566, #15250, #37926, #21902, #14801, #29929, #36097, #22349, #43657, #15720, #58814, #43205, #87201, #1499, #87657, #7674, #51677, #57884, #66832, #29473, #44581, #8142, #88122, #36558, #65017, #73932, #73484, #50297, #30861, #65939, #28998, #8596, #79203, #65473, #80111, #30383, #59755, #44110, #37473, #37025, #66383, #1969, #45032, #73013, #21423, #59276, #591, #14346, #9048, #23280, #117, #72106, #58361, #52154, #1050, #86740, #52607, #39318, #82434, #25597, #10452, #46894, #16636, #68236, #54480, #81489, #2897, #83349, #40254, #17584, #75336, #45490, #54019, #75795, #18042, #81953, #90440, #24199, #89512, #74391, #60211, #38864, #82886, #9519, #89050, #18497, #10918 ),
 ( #61606, #74881, #38407, #47361, #61154, #23744, #4297, #3357, #2446, #89989, #67316, #53076, #24677, #3839, #33177, #60674, #32247, #25143, #39786, #69170, #76276, #53562, #88595, #68709, #17110, #11402, #31324, #32721, #45974, #9991, #67770, #31780, #46433, #18985, #26065, #12836, #55906, #92811, #77685, #20394, #83831, #41674, #27976, #54954, #70122, #56866, #13764, #84758, #48779, #47837, #27487, #49265, #85247, #55439, #63970, #91396, #63032, #76739, #33644, #12336, #56381, #11866, #62554, #85708, #78160, #49724, #26551, #84291, #41182, #78621, #19906, #19441, #20853, #42612, #6663, #40717, #5259, #71529, #62066, #69635, #48307, #91863, #4763, #90900, #13298, #70592, #27017, #42136, #71054, #77206, #34128, #5719, #34594, #63503, #92332, #6186, #35053, #38172, #21318, #64912, #86629, #67087, #66615, #15, #14241, #51923, #28893, #2220, #23979, #46213, #31561, #16416, #60453, #7123, #37709, #35993, #52853, #82207, #57782, #17362, #31104, #38649, #23045, #28432, #80813, #88375, #15962, #45269, #67553, #2682, #16879, #44816, #81731, #45738, #1738, #74649, #89288, #75117, #23525, #52394, #35539, #73719, #59991, #8830, #88830, #9775, #79089, #64454, #24441, #53322, #93280, #57325, #30625, #86167, #50189, #74172, #43099, #59526, #81271, #72004, #9289, #25376, #60915, #33412, #69404, #68007, #54715, #76979, #68950, #48545, #10227, #11173, #68475, #24923, #39094, #61395, #40034, #76044, #76517, #90227, #4081, #19217, #83593, #47614, #89761, #91152, #40954, #46669, #32952, #3611, #55213, #11640, #3136, #17816, #32016, #40487, #91638, #53800, #83126, #75573, #18756, #47131, #61844, #82668, #69875, #4536, #84528, #90676, #62311, #10695, #25836, #84067, #26318, #48075, #5014, #54256, #12109, #33896, #62803, #39552, #18277, #26792, #32497, #55678, #19676, #6418, #49034, #70368, #84998, #78390, #92565, #28207, #57551, #85935, #77930, #49956, #20153, #242, #85483, #6895, #64221, #50433, #63739, #27258, #36221, #78848, #12590, #86875, #57095, #13073, #13995, #41436, #41909, #13530, #86396, #22029, #49500, #21085, #93051, #71772, #58020, #43330, #42379, #29123, #28664, #70822, #77445, #72227, #35769, #63271, #5493, #56633, #14472, #42857, #34366, #92103, #64682, #71292, #7341, #93508, #21548, #56145, #79337, #65141, #5954, #20630, #34827, #27737, #35294, #37601, #14924, #16310, #38060, #74061, #44239, #52739, #80240, #51809, #72679, #22476, #1174, #45162, #43777, #51348, #16770, #66968, #38546, #15377, #73150, #30056, #67449, #8724, #8274, #74528, #9662, #89181, #29605, #58938, #31455, #45624, #7798, #37154, #80703, #36683, #50898, #2108, #66511, #15854, #30998, #59885, #65606, #87327, #1632, #87788, #719, #2577, #66062, #58483, #52286, #22938, #44712, #73613, #81166, #30513, #59409, #60344, #79782, #9181, #88264, #23421, #88725, #23873, #81621, #10125, #25274, #53699, #83481, #32847, #46109, #90123, #67904, #76873, #90568, #53210, #33783, #68844, #31913, #25726, #82089, #24815, #54151, #33305, #62698, #83020, #61736, #39925, #18638, #4898, #83966, #18172, #69767, #69299, #82566, #40848, #19114, #76412, #38991, #17249, #3495, #55098, #3972, #75013, #3027, #54610, #47025, #47969, #47506, #11534, #60805, #40381, #12000, #89644, #32388, #24333, #17714, #75928, #11055, #46567, #4427, #62203, #91033, #75466, #26203, #10587, #39450, #68367, #61288, #41806, #56991, #55574, #91995, #57448, #78744, #79221, #56034, #27148, #70717, #14364, #49397, #63165, #21443, #50316, #36116, #70259, #5849, #72124, #86289, #19570, #84889, #92459, #84422, #91528, #13887, #13426, #27623, #42741, #6790, #48437, #34258, #78288, #34720, #41322, #43224, #20039, #12474, #92944, #77340, #48917, #77818, #28104, #56520, #12967, #7240, #26685, #85829, #85379, #5393, #63634, #20528, #6313, #42273, #71184, #35181, #20980, #64105, #49847, #71656, #35665, #64580, #93405, #28557, #34910, #14998, #6507, #21637, #78930, #65218, #78474, #42945, #6038, #93587, #56230, #92655, #93130, #7420, #7876, #64305, #35845, #14080, #86472, #72755, #58107, #28285, #43857, #43405, #27826, #36766, #86953, #50516, #78015, #85092, #71374, #29207, #71852, #49118, #20241, #6972, #86016, #22105, #64762, #79414, #13155, #28746, #50975, #41991, #35386, #79859, #92188, #21166, #57629, #70904, #14549, #72300, #36302, #85561, #323, #56715, #57176, #63821, #20709, #42464, #27343, #49579, #13611, #50035, #54122, #54581, #30134, #1252, #15935, #83453, #23497, #37232, #90540, #25699, #11505, #44326, #44789, #47472, #32817, #87405, #59018, #66587, #58564, #65687, #82993, #81240, #1708, #18143, #75900, #22552, #8349, #52365, #73690, #15455, #18607, #87865, #80315, #67052, #51426, #23014, #51893, #3464, #30591, #80786, #61707, #76379, #32359, #59493, #801, #66137, #8800, #74142, #73238, #88346, #37679, #61259, #9260, #16387, #45237, #46997, #38137, #90094, #25246, #11024, #29681, #39893, #68814, #3944, #13394, #26652, #83934, #92911, #12936, #69271, #49816, #41776, #34228, #55065, #19540, #70686, #4400, #20495, #77788, #63134, #11970, #33279, #47940, #41292, #55542, #84857, #19086, #84391, #4869, #5816, #27592, #78713, #35150, #20009, #64071, #40818, #70227, #69737, #56488, #85797, #33751, #20948, #34690, #42237, #48406, #62174, #77309, #91963, #62663, #48887, #71150, #6279, #49362, #91497, #85347, #78256, #5362, #28073, #56960, #40354, #27118, #56002, #91006, #12444, #63604, #92428, #26174, #76843, #57419, #13855, #1039, #66370, #73471, #1488, #65004, #64550, #52144, #51209, #28524, #57873, #7212, #37461, #71626, #28985, #93374, #37013, #73001, #6759, #58348, #80552, #72540, #42710, #35633, #14789, #72095, #86258, #21409, #106, #43644, #79647, #80100, #86727, #7659, #22796, #87189, #15239, #50284, #29917, #44568, #79190, #36544, #36085, #58801, #44095, #14334, #43194, #21891, #8129, #30371, #50763, #65460, #576, #22338, #29460, #65927, #87646, #8583, #51663, #88110, #15707, #59262, #23266, #45962, #32233, #17096, #38850, #75783, #2432, #17572, #82874, #67304, #73920, #31312, #67758, #16625, #60661, #18027, #46881, #61141, #74378, #89977, #25131, #74869, #54007, #10903, #25582, #2884, #31769, #81024, #45479, #82422, #89036, #10439, #39305, #30849, #16168, #68222, #39771, #68695, #3826, #38394, #37915, #45020, #24663, #1956, #60198, #9506, #32707, #9037, #24186, #66819, #3342, #46421, #59742, #89498, #61593, #9979, #88584, #23732, #81939, #53064, #52595, #81476, #53549, #75322, #90426, #27003, #11850, #84277, #63488, #5244, #91849, #11388, #41661, #85230, #90887, #19428, #18969, #5703, #55891, #83335, #62052, #76260, #84745, #42121, #92794, #33628, #26050, #63017, #91379, #26536, #47344, #20380, #19892, #35040, #77193, #48763, #18481, #48290, #34579, #12322, #41166, #49251, #69620, #77669, #12821, #70104, #69155, #62538, #70578, #40240, #92319, #27473, #34115, #54937, #4283, #83816, #55424, #4748, #56366, #33161, #78146, #47822, #13284, #71038, #63954, #6172, #54465, #76724, #40700, #28878, #28418, #43991, #73365, #57309, #8478, #22234, #21782, #42596, #7106, #461, #56851, #8012, #65354, #50657, #93264, #20838, #35524, #57766, #43083, #72436, #6645, #71988, #86151, #58241, #15128, #37357, #22682, #7554, #51555, #21302, #86612, #50175, #72888, #66264, #79071, #27961, #51105, #29810, #14223, #49708, #35977, #79544, #64897, #36439 ),
 ( #78604, #85692, #29350, #71511, #14442, #14684, #80443, #13748, #43539, #64438, #79991, #87085, #36906, #65823, #931, #58691, #87534, #15588, #44461, #59634, #16063, #30261, #52493, #31208, #67193, #67654, #81370, #60093, #10332, #45849, #38750, #52034, #82313, #32127, #37810, #88932, #88480, #46313, #2780, #59153, #8932, #23150, #31661, #82769, #39659, #74273, #66717, #9874, #38280, #2328, #87997, #61023, #60553, #75673, #24081, #89391, #80918, #52956, #75218, #81834, #16984, #89869, #16519, #24545, #53429, #74755, #39199, #25029, #1379, #17463, #68111, #44917, #23627, #3237, #9396, #53901, #17921, #73819, #1845, #46772, #10798, #30732, #45370, #25939, #25479, #13170, #12210, #83232, #18861, #61943, #92203, #32603, #83699, #54358, #91739, #33999, #61493, #19316, #41541, #33513, #68582, #3718, #69508, #33053, #18378, #90325, #54821, #4639, #40594, #41055, #47718, #62419, #77550, #48178, #69981, #47236, #55778, #5593, #11281, #91261, #90780, #19779, #5122, #76148, #40134, #69051, #62902, #56247, #4180, #76618, #11741, #77079, #26425, #55317, #84168, #34467, #26891, #49134, #84631, #48650, #12701, #70465, #63373, #27359, #85108, #20258, #78030, #72316, #14564, #35861, #56731, #21181, #43421, #70922, #22119, #79428, #64778, #13628, #34925, #49594, #42961, #57191, #86491, #20724, #86032, #6523, #7437, #29225, #51440, #36782, #21654, #65703, #42479, #71867, #71391, #58121, #87418, #35401, #22566, #36319, #43872, #28301, #63839, #50052, #93603, #64321, #50531, #72769, #7893, #50988, #93146, #86966, #79873, #78947, #65233, #78490, #14097, #6988, #338, #15013, #80328, #815, #29695, #58579, #28761, #57644, #42006, #6053, #92670, #27842, #85576, #9759, #17345, #1721, #8364, #30607, #67069, #44802, #88815, #46196, #75101, #89273, #8812, #60437, #24423, #45251, #53305, #10211, #53785, #2204, #31088, #15470, #73703, #16863, #23509, #38634, #67537, #59030, #44341, #2666, #67993, #39079, #3121, #66599, #66148, #73252, #52837, #30147, #59509, #37693, #32001, #37245, #88359, #1265, #31545, #74631, #87877, #59976, #82191, #74156, #23028, #51907, #16400, #52378, #80799, #15947, #81255, #9272, #38154, #81713, #23963, #45721, #60897, #89746, #24907, #39539, #69861, #19663, #25362, #47599, #47116, #33881, #84054, #17802, #90213, #10681, #55199, #70355, #27245, #61828, #54242, #91136, #25821, #54701, #75559, #48531, #26304, #63258, #11625, #76965, #46655, #76501, #62790, #18740, #40471, #77432, #4066, #19201, #48061, #69388, #3594, #90661, #12094, #68460, #91625, #40941, #4521, #83112, #32483, #18263, #83577, #12575, #4998, #61380, #76028, #33397, #41423, #62296, #11157, #40018, #26778, #55664, #5481, #84516, #34353, #68935, #92089, #82653, #32936, #64208, #86862, #7786, #49944, #42843, #20139, #21536, #43318, #79323, #49488, #58007, #85471, #57083, #77919, #27722, #6406, #50418, #49022, #56620, #22017, #72214, #43766, #20618, #78378, #35280, #72667, #13983, #13519, #79768, #14911, #707, #34815, #93038, #36672, #50887, #13061, #42367, #85922, #41897, #56132, #7330, #71759, #21073, #36210, #65129, #70811, #92553, #6884, #28194, #5943, #65593, #71279, #63728, #57542, #78837, #35757, #64670, #86385, #93498, #28651, #84985, #14461, #231, #29111, #46094, #30044, #58925, #38045, #15364, #30501, #87775, #88711, #66954, #51335, #1617, #9646, #2093, #22925, #30983, #66049, #74999, #37588, #52725, #16296, #2562, #15841, #73134, #82074, #59871, #58470, #38978, #74048, #37141, #23859, #87314, #51795, #59395, #38532, #67890, #88248, #81608, #45149, #16757, #10111, #89168, #23406, #29591, #74513, #80686, #22461, #24319, #44698, #45611, #67435, #52273, #44225, #8710, #31441, #80228, #60331, #53196, #81152, #1161, #8260, #73599, #9167, #66499, #17232, #75453, #18157, #61272, #33291, #83949, #12458, #91512, #76396, #26668, #68352, #3958, #3480, #19101, #48420, #32372, #77326, #91018, #4882, #83005, #89629, #47011, #54595, #90107, #11519, #33766, #62678, #76857, #25259, #47954, #11983, #32831, #40832, #55558, #41306, #83466, #18622, #3013, #54136, #4413, #11039, #26187, #55080, #46552, #31899, #69751, #84406, #19555, #60791, #75914, #53683, #24798, #40366, #17700, #39908, #68829, #82551, #10572, #61722, #39436, #90553, #62188, #25712, #47487, #69283, #35166, #16081, #70243, #71169, #34706, #84873, #5376, #27607, #6297, #42255, #44007, #56505, #64088, #80459, #22251, #15146, #27133, #58708, #8494, #12953, #92928, #63619, #22698, #72905, #34243, #77803, #91980, #8029, #59169, #63149, #49380, #41791, #80007, #13412, #28089, #56016, #37372, #36926, #52053, #58258, #65840, #20024, #87101, #51573, #51121, #948, #48901, #70702, #5833, #29826, #88015, #92444, #78273, #85363, #87551, #15607, #44479, #20512, #66282, #73384, #80936, #1395, #30279, #23170, #52976, #46332, #24097, #17001, #61043, #38299, #60573, #2797, #81851, #1861, #2347, #31679, #73835, #75235, #89409, #45869, #52511, #8949, #88498, #88950, #67214, #9892, #59654, #31225, #45388, #24563, #82331, #17938, #89886, #38767, #32144, #81387, #74775, #16535, #17481, #82786, #74289, #46789, #53450, #68130, #60110, #37828, #67671, #10349, #9413, #39215, #3254, #25046, #53918, #44934, #66734, #30752, #23645, #15922, #30579, #74126, #87393, #51412, #35831, #310, #37218, #43841, #59004, #87853, #79400, #64746, #23001, #88331, #1696, #23484, #86940, #86458, #93573, #73223, #50501, #79845, #29191, #59475, #28730, #50962, #21617, #51878, #1239, #57615, #80304, #8788, #785, #14536, #43391, #36750, #58089, #72285, #7406, #22092, #65673, #7863, #8337, #14985, #29668, #44777, #15444, #66125, #36287, #80772, #66574, #65206, #58548, #72742, #73677, #30121, #52351, #22540, #81227, #37666, #44311, #16373, #45224, #61354, #88788, #2174, #82160, #39991, #53761, #59948, #67037, #82627, #3091, #68907, #24880, #90188, #31061, #17775, #4039, #23936, #17318, #32911, #54675, #31976, #89713, #52808, #68432, #25336, #32452, #2642, #11125, #38608, #10185, #81686, #74601, #53276, #3563, #16835, #9731, #61800, #54215, #90631, #67512, #31520, #46170, #25793, #60869, #60408, #83548, #18707, #47571, #45692, #75073, #9247, #38125, #89246, #24399, #39054, #67966, #46630, #83084, #75530, #10654, #18239, #47091, #39511, #75995, #63230, #55637, #26272, #28169, #4969, #91104, #77890, #62269, #12066, #33853, #13035, #12542, #40913, #42340, #71252, #41870, #70326, #93011, #76938, #69833, #84958, #55167, #77405, #62763, #70783, #20109, #4492, #48505, #56590, #48989, #91596, #5916, #19175, #57059, #84488, #34786, #92062, #49463, #26751, #84030, #35253, #63701, #11596, #85895, #27216, #48033, #92527, #40444, #19636, #41392, #85444, #21047, #5456, #27693, #56103, #20593, #76476, #78351, #13493, #69361, #6381, #34324, #33368, #64178, #79290, #66470, #15812, #8233, #35730, #42813, #29084, #80657, #677, #6855, #13956, #29561, #43738, #44670, #65564, #37111, #71728, #58442, #73571, #64643, #57975, #8680, #1587, #72638, #36643, #93471, #15338, #66020, #73105, #43289, #51767, #14432, #50860, #28624, #21509, #201, #44199, #57513, #50387, #37558, #1132, #30469, #72186, #7302, #86828, #59365, #7758, #36182, #88217, #49915, #78810, #86358, #21986, #65101, #79742, #14884, #87288, #22434, #51307, #80199, #30014, #58898, #87744, #22896, #32340, #16266, #59839, #10080, #2532, #66923 ),
 ( #3445, #31868, #23829, #89598, #88680, #39874, #31410, #46522, #38948, #90076, #9612, #2061, #75880, #24769, #52241, #32800, #67858, #30951, #53651, #81123, #52692, #24287, #61241, #61689, #89136, #60757, #82521, #45116, #25228, #17669, #46062, #81573, #74018, #16721, #53162, #38499, #2983, #45576, #67404, #74481, #75423, #10540, #23373, #18126, #39406, #46979, #60299, #82044, #17201, #68321, #68794, #74967, #3924, #54101, #82973, #11005, #9135, #38012, #48388, #26153, #70210, #27570, #56467, #70668, #83915, #41756, #5797, #26633, #63585, #20477, #35130, #77291, #12421, #90520, #55047, #91943, #4848, #19987, #48864, #40337, #54563, #77769, #49344, #78238, #13376, #47922, #47453, #83431, #34210, #11487, #40800, #19067, #42218, #18587, #11951, #76361, #12917, #55984, #69253, #41272, #92410, #55523, #4381, #33259, #91482, #76825, #62156, #90985, #69717, #84372, #62644, #63115, #33732, #19521, #71132, #5343, #27097, #84838, #6261, #1025, #6743, #28970, #28507, #15225, #65444, #92895, #71608, #85781, #36528, #51650, #8569, #43177, #35616, #72524, #7195, #36070, #56944, #29903, #7644, #44555, #86709, #58332, #28054, #57855, #44081, #90, #21874, #58787, #79170, #559, #29443, #50748, #78697, #72079, #64987, #87175, #22324, #13838, #64052, #51195, #22781, #87631, #80536, #21392, #20931, #49800, #80082, #42689, #14317, #57399, #15690, #64531, #79632, #93356, #72983, #8113, #86241, #14774, #37000, #43627, #50262, #65912, #73458, #1938, #52130, #66357, #88572, #67291, #9490, #9967, #23720, #2420, #46409, #81927, #74855, #88093, #24646, #68211, #73908, #31300, #30833, #82410, #38839, #1472, #45006, #59247, #67746, #25120, #75772, #16612, #9024, #45947, #74367, #38377, #30358, #3330, #2872, #18015, #60186, #31756, #23251, #89024, #17557, #24171, #53052, #32220, #52583, #60648, #89486, #17079, #81011, #45467, #53534, #16155, #75309, #10428, #39292, #37903, #66808, #59730, #61127, #81463, #89966, #53994, #82863, #46868, #37448, #91834, #20363, #5689, #84264, #34563, #76245, #11836, #11377, #26988, #56350, #40227, #85212, #5229, #12805, #90873, #3815, #26037, #62521, #69143, #19414, #41647, #63472, #84730, #4271, #55878, #19879, #40687, #48750, #92301, #49235, #91362, #26523, #10892, #33149, #12309, #62039, #27458, #68681, #54920, #61582, #34102, #70086, #32696, #55411, #77654, #69605, #39755, #90414, #4735, #83800, #25571, #54451, #18955, #33613, #76710, #77179, #47809, #48277, #83324, #41153, #63004, #18470, #47329, #15113, #20824, #43067, #42581, #29331, #79530, #13269, #85676, #6153, #50640, #65805, #22667, #57294, #49694, #86595, #21285, #50158, #71021, #43972, #21765, #58676, #7090, #72422, #42106, #71972, #58224, #14207, #35962, #72873, #93249, #14669, #43524, #64881, #92777, #86136, #7538, #35025, #87069, #36423, #93707, #78589, #63939, #13728, #79056, #28402, #28862, #56836, #57749, #71496, #65340, #445, #87521, #7997, #22217, #36890, #6627, #51087, #35507, #79975, #29796, #64423, #78131, #917, #27945, #37795, #44445, #66702, #9382, #80902, #31194, #82297, #17447, #31647, #44901, #2765, #60537, #81354, #89375, #46297, #89853, #38264, #67177, #51540, #16049, #52942, #59615, #74738, #9859, #1364, #80429, #38733, #10316, #75201, #39184, #8918, #8463, #15575, #88916, #66249, #1830, #24531, #16504, #73351, #37343, #52480, #73804, #30247, #59137, #30717, #45356, #23613, #24066, #88466, #74258, #53413, #2310, #81819, #87981, #67639, #68096, #23133, #60079, #16968, #3221, #45834, #52016, #32111, #61008, #91246, #12684, #63357, #4165, #32588, #33496, #61927, #90764, #17904, #84615, #62404, #5578, #47703, #19301, #53885, #83684, #69965, #54806, #76602, #19764, #40119, #55300, #26410, #18845, #39643, #33037, #84153, #82752, #5106, #48161, #11725, #90309, #46758, #61479, #25923, #69035, #69492, #3703, #40578, #83217, #77064, #12194, #34449, #48632, #4623, #77534, #25462, #41037, #54342, #33984, #70451, #18362, #25014, #62887, #26875, #11266, #75658, #91722, #55762, #47222, #41525, #10782, #68567, #76132, #18546, #70171, #34175, #55007, #5305, #19953, #63547, #76788, #40763, #25191, #83396, #26596, #33222, #48352, #77255, #68757, #54064, #12385, #77731, #84803, #12881, #76323, #75843, #82935, #62603, #39834, #69216, #47414, #48824, #18087, #40301, #10966, #41231, #84335, #46941, #69681, #90486, #3888, #32765, #26113, #4345, #4811, #61653, #62118, #11449, #55486, #63077, #34637, #41719, #33692, #70635, #25644, #83879, #54527, #91907, #5763, #90949, #19030, #19486, #27061, #47884, #11914, #91445, #55948, #28019, #72049, #29411, #58301, #72495, #85750, #43599, #7611, #28476, #36499, #87145, #36969, #50233, #14285, #92376, #56910, #58, #6710, #21841, #50717, #42182, #27535, #79603, #51166, #22295, #80053, #49769, #49308, #56428, #36040, #13341, #42657, #20897, #15193, #85290, #13805, #78202, #14744, #57825, #20439, #43145, #65416, #57369, #71095, #6228, #93324, #78664, #35098, #64016, #71574, #86211, #64498, #64957, #35583, #21363, #526, #7165, #28939, #92856, #44053, #72954, #79136, #86676, #8081, #17050, #67259, #991, #73429, #87599, #38346, #53502, #10397, #44977, #8539, #74337, #8996, #37874, #58757, #31727, #9460, #46378, #88542, #60156, #29873, #30800, #45916, #1910, #23691, #60618, #80983, #2391, #31269, #59699, #80507, #73878, #88995, #22745, #74822, #24142, #52555, #89456, #16126, #53020, #81898, #81431, #15655, #66780, #9937, #51620, #38811, #67715, #16580, #37418, #44525, #66329, #45436, #2845, #24616, #1442, #82378, #30327, #17528, #75278, #65882, #59217, #88062, #23219, #52099, #40198, #39725, #55383, #84704, #68649, #19851, #33583, #41126, #25542, #32189, #54423, #90844, #3783, #18925, #70057, #5199, #19385, #32666, #84235, #48249, #69115, #77151, #34072, #77625, #26006, #54890, #39262, #61553, #40657, #47298, #62491, #91331, #82831, #68177, #26493, #91808, #62974, #26960, #90387, #89934, #3299, #76681, #53964, #83294, #18441, #55851, #61095, #76215, #25090, #12281, #4705, #17984, #83769, #48723, #4240, #46836, #75738, #33120, #11344, #10863, #62009, #47779, #11806, #69576, #79025, #63913, #42551, #21736, #57264, #50126, #63443, #93678, #43496, #49204, #71468, #70993, #57720, #14178, #41616, #20334, #34535, #43040, #415, #51058, #85647, #78100, #21256, #49666, #78561, #5660, #72392, #71942, #87040, #35477, #7063, #70537, #6599, #86567, #64394, #93220, #86107, #7509, #36394, #50612, #6125, #79502, #14638, #28373, #65307, #29301, #12774, #35933, #64851, #92274, #34996, #28836, #20795, #58196, #22190, #56321, #27430, #85185, #13241, #42077, #92747, #27918, #56805, #13699, #23587, #887, #30219, #73325, #9834, #43944, #1337, #36862, #9351, #45331, #72841, #30688, #52914, #44874, #24504, #79946, #80876, #44417, #29770, #15084, #37315, #16023, #51986, #52454, #66223, #73776, #88890, #59587, #81328, #65778, #67149, #16941, #22640, #8891, #8436, #31166, #16475, #7969, #87490, #58648, #74232, #67614, #51512, #59110, #80400, #88438, #23105, #37769, #15546, #45804, #38236, #60513, #66674, #2283, #87952, #1802, #60052, #24038, #81793, #74713, #38707, #2742, #31622, #89348, #68071, #32564, #25897, #82270, #33472, #90739, #76108, #24989, #46272, #60981, #54316, #68539, #4142, #32080, #3678, #17880, #83657, #40552, #62865, #48137, #33013, #77040, #53862, #83191 ),
 ( #54779, #33961, #11240, #47677, #17423, #18339, #4599, #47194, #40095, #12171, #61456, #18820, #76578, #69011, #3196, #90287, #11701, #75176, #62375, #69467, #61904, #82728, #10289, #89828, #91219, #25438, #26386, #46732, #55274, #75635, #84129, #19279, #91698, #41014, #69937, #5080, #10758, #53386, #39615, #39159, #72278, #56207, #7397, #21144, #28722, #13134, #19740, #41970, #78453, #85066, #6482, #57607, #86450, #6950, #20218, #71831, #35823, #56693, #64737, #21608, #65199, #13589, #42441, #26850, #49095, #28265, #34889, #50014, #78907, #70430, #55738, #14054, #79391, #50490, #14528, #77994, #77508, #84590, #64281, #41501, #70883, #6014, #43383, #48608, #63800, #12656, #42918, #85994, #5556, #71351, #93565, #85540, #34426, #63333, #27801, #92629, #92164, #27321, #20688, #49558, #35360, #93110, #57154, #36279, #9239, #44769, #37658, #50954, #81220, #32322, #36742, #58996, #58541, #45217, #1688, #59467, #16366, #23476, #87386, #2165, #29661, #1231, #22084, #65664, #44302, #88321, #58079, #777, #61224, #74119, #82954, #22533, #51405, #73211, #18109, #51869, #80297, #25211, #54084, #39856, #72735, #8328, #75863, #90058, #79837, #15436, #30113, #86931, #302, #38118, #15913, #87844, #67028, #46961, #14977, #37210, #80762, #66117, #43833, #10986, #22994, #7855, #30569, #73669, #8780, #66566, #52343, #29182, #33242, #34653, #63567, #34193, #62625, #85310, #69235, #4364, #77274, #54546, #69700, #62137, #63097, #12403, #90504, #40782, #48844, #41251, #90968, #70192, #11469, #20458, #76807, #91925, #55506, #41738, #55029, #18568, #27553, #5325, #3907, #78220, #19504, #76343, #27080, #32784, #26134, #4829, #77749, #13359, #33713, #55967, #84355, #84820, #49326, #92393, #91464, #68778, #19969, #83898, #61672, #56448, #12900, #83414, #25665, #47905, #5779, #48372, #47434, #40320, #70651, #26615, #19049, #11933, #541, #64033, #21857, #72966, #6244, #50246, #8095, #87612, #36053, #28952, #35113, #78680, #7178, #6726, #87158, #43611, #71114, #49783, #92875, #14757, #29886, #80519, #21376, #13820, #50731, #79152, #14300, #28037, #36982, #79615, #22762, #64971, #36512, #56926, #74, #22307, #72061, #57838, #65894, #57383, #72507, #7627, #86692, #85764, #43160, #65427, #20914, #51178, #29424, #58314, #42672, #71589, #35598, #80065, #86226, #15208, #64513, #44065, #93339, #1006, #58770, #51633, #42200, #28490, #10412, #80996, #16595, #16138, #31739, #61110, #44990, #89949, #9951, #17541, #1922, #8552, #30816, #67274, #73891, #89008, #46393, #75293, #89469, #9008, #60632, #24630, #45451, #53517, #39276, #53978, #2404, #31284, #15672, #37887, #17063, #23704, #38823, #67730, #59231, #44539, #2857, #68194, #3314, #32203, #66792, #66341, #73442, #53035, #30341, #59713, #88556, #25104, #37432, #52567, #1455, #82393, #74838, #88077, #60170, #23233, #74351, #52113, #81447, #9474, #38360, #24155, #81911, #45930, #18938, #54905, #55396, #40212, #47793, #91820, #33598, #26506, #39739, #70072, #19865, #76695, #83784, #84248, #69128, #11821, #26973, #62506, #19399, #68663, #5213, #48735, #25556, #40672, #47313, #34086, #48262, #17999, #90399, #10876, #77164, #70550, #27443, #62024, #54436, #91346, #26022, #69590, #75755, #77639, #12294, #63456, #4720, #41139, #46852, #62989, #55864, #84716, #12790, #41630, #4256, #5673, #34548, #92286, #3799, #90858, #82847, #32680, #61566, #83309, #18454, #76229, #11359, #33134, #57279, #71480, #7075, #35009, #6612, #20808, #86580, #43510, #65792, #51074, #35948, #79962, #27929, #86121, #56819, #72408, #7983, #85661, #36877, #50626, #58210, #42564, #49219, #35492, #14192, #49679, #64867, #87055, #22204, #36409, #78574, #7524, #65324, #21270, #429, #15099, #902, #43053, #71957, #56335, #13712, #57735, #64407, #79516, #14654, #6137, #85197, #29317, #43959, #72858, #20347, #93234, #13254, #78115, #93693, #71006, #28387, #50142, #42091, #63924, #79040, #92762, #28849, #21750, #87507, #74245, #2754, #88452, #68084, #29784, #30703, #87968, #44432, #58663, #80888, #22654, #23119, #31180, #37782, #52927, #81806, #73338, #51527, #16955, #82285, #89361, #17436, #16036, #80416, #15561, #67164, #8449, #73789, #52002, #53400, #37328, #44887, #66236, #45820, #88903, #1351, #9367, #31635, #23599, #30234, #59124, #59602, #8905, #66689, #1817, #52467, #81341, #16489, #2297, #45344, #38251, #38720, #60065, #24053, #74726, #9847, #60525, #67626, #24519, #46286, #75190, #10303, #39173, #10771, #25004, #69480, #84603, #41515, #76121, #39631, #11713, #40108, #69023, #89842, #62876, #40566, #77521, #25910, #91234, #32095, #61916, #48149, #33025, #54793, #91710, #18352, #33485, #4611, #90752, #17894, #11253, #62391, #60997, #77053, #26399, #83672, #68555, #53875, #3692, #4155, #47210, #47689, #75648, #18834, #61470, #55287, #84141, #12673, #26862, #76591, #55750, #32577, #19290, #90300, #12182, #48620, #25452, #3209, #41025, #5093, #83205, #82741, #69951, #33972, #54331, #19753, #46747, #7409, #50504, #63811, #21622, #79402, #6494, #14538, #65208, #14987, #28276, #86006, #70441, #49569, #78005, #78918, #13600, #42452, #63345, #36289, #14067, #50964, #93120, #64750, #5568, #35375, #43393, #64294, #57166, #312, #85552, #6961, #42932, #21155, #85080, #78464, #71841, #34439, #72287, #35834, #50025, #41981, #92177, #13145, #71364, #20699, #93576, #49108, #28734, #34900, #57618, #86461, #79847, #29195, #58092, #86942, #70894, #22094, #6026, #27333, #56220, #92643, #20231, #27815, #56705, #30124, #36754, #59007, #1698, #73227, #23487, #74606, #9735, #23939, #37220, #88791, #52811, #73679, #81690, #38612, #82165, #30581, #59482, #43845, #8339, #45227, #51882, #67041, #2178, #87395, #72744, #31064, #2645, #67515, #31523, #1242, #788, #7865, #81230, #58551, #87855, #66127, #60411, #65676, #23004, #29670, #59952, #9250, #22542, #88335, #16839, #8790, #51415, #80307, #44779, #80775, #15446, #44315, #15925, #37669, #66577, #16377, #52354, #74131, #45695, #38128, #89250, #24402, #53281, #48038, #53764, #75999, #75534, #62273, #18712, #46173, #24883, #39057, #83553, #4972, #69838, #47575, #75077, #26756, #61804, #82630, #76480, #10188, #17779, #18242, #26277, #55641, #83088, #54679, #32914, #11603, #91600, #76943, #47094, #62768, #91108, #46633, #33858, #12070, #69366, #3095, #67969, #90191, #40917, #90636, #31979, #60872, #25798, #11130, #17322, #40448, #4496, #89719, #33374, #10658, #39514, #25339, #68435, #3567, #39994, #4044, #32457, #55172, #84033, #19178, #61357, #54219, #68913, #85449, #12547, #56108, #34791, #49920, #48508, #84962, #50394, #71735, #72193, #48995, #20113, #63706, #7310, #42346, #77894, #14439, #43296, #29091, #63236, #92531, #65108, #79299, #41397, #13038, #20597, #77409, #84494, #6861, #6386, #49467, #35736, #93478, #70331, #27221, #71257, #27697, #34330, #36189, #41875, #5460, #85901, #92067, #70786, #5921, #21053, #78357, #56595, #210, #19640, #78816, #13497, #35257, #64183, #93015, #28173, #57063, #13962, #42820, #64649, #28631, #57520, #86364, #21516, #66479, #58450, #30478, #686, #74491, #66029, #81132, #44678, #30961, #44206, #7766, #1141, #16276, #73580, #59849, #73113, #36651, #16733, #59374, #86837, #67414, #8689, #65572, #88226, #21994, #87295, #58906, #66932, #2543, #30023, #1596, #37568, #52251, #38510, #23838, #87752, #9623, #9145 ),
 ( #50867, #23382, #45127, #74028, #51314, #88690, #22441, #22904, #79749, #29570, #8240, #38022, #14891, #80206, #52704, #2070, #45587, #15345, #37120, #51776, #57984, #15821, #80665, #81585, #43745, #72645, #10090, #75434, #11963, #90997, #53175, #24779, #32352, #24298, #69728, #18599, #46990, #61251, #47465, #40347, #82054, #67870, #18136, #10552, #74978, #76836, #53662, #46072, #32810, #17211, #60768, #82531, #61700, #90087, #89609, #26166, #55058, #90532, #25239, #47933, #31879, #17680, #39886, #38958, #54113, #46532, #25692, #68807, #2993, #3457, #11498, #3936, #39417, #54574, #68334, #40811, #83927, #31422, #82986, #75891, #60311, #19079, #11016, #83445, #76372, #69264, #89149, #4393, #33270, #62167, #42229, #35140, #62656, #77302, #34682, #55994, #84384, #43974, #34220, #19533, #85337, #55535, #41283, #63126, #20488, #77780, #70219, #58226, #87071, #49354, #41768, #15115, #12433, #5354, #27581, #48399, #48876, #91955, #78248, #56478, #91490, #12927, #6272, #13386, #27110, #71143, #84849, #72875, #19998, #64063, #5808, #92904, #70678, #63596, #51089, #28064, #33743, #7999, #92420, #22219, #79977, #26645, #4860, #90371, #4687, #6457, #61539, #33102, #11329, #83753, #70034, #55364, #25527, #41104, #40639, #25075, #12260, #84216, #47764, #75265, #82363, #68633, #26475, #40180, #46364, #53487, #69099, #83279, #19364, #4226, #76662, #17512, #61992, #48228, #10380, #3766, #77130, #35332, #18423, #76200, #39247, #54872, #11789, #18909, #82816, #91313, #53948, #54406, #68163, #61077, #39709, #69558, #3283, #89919, #89440, #33561, #24598, #17967, #46820, #32651, #32176, #47283, #75722, #10845, #62471, #90827, #25987, #1211, #28242, #72259, #30093, #15893, #58058, #50933, #57129, #29641, #51385, #87364, #57585, #66099, #93541, #65177, #85971, #35801, #14507, #58520, #21121, #64714, #58976, #80276, #51848, #28700, #86429, #43363, #80742, #22065, #21586, #87825, #22976, #8761, #42892, #7376, #44750, #73651, #49989, #50467, #282, #78884, #64258, #15415, #79817, #29161, #44282, #73190, #14031, #6928, #14958, #36257, #71806, #93088, #79370, #86910, #65642, #43813, #72713, #7836, #756, #36723, #22514, #8309, #37192, #3065, #31493, #54187, #38100, #67009, #46145, #23457, #38581, #2145, #31950, #75049, #59448, #9700, #17749, #10160, #31034, #39029, #74100, #83057, #45664, #60843, #24371, #10626, #23909, #81201, #90161, #67942, #66547, #47061, #82131, #45197, #89685, #1668, #59924, #67484, #46602, #75966, #2615, #24852, #53250, #53736, #18211, #3534, #60381, #37639, #82602, #88763, #30551, #32424, #75504, #52324, #88300, #16807, #68406, #17288, #16347, #9219, #39484, #89220, #61323, #25309, #52780, #81659, #74571, #19148, #34293, #91564, #77855, #91073, #54646, #63671, #77375, #39961, #20562, #55608, #18676, #12513, #68877, #11567, #12038, #20078, #49434, #76908, #48475, #26721, #5428, #85414, #70752, #40885, #56560, #56073, #40415, #27663, #5886, #63201, #90603, #4007, #84000, #41841, #84457, #61770, #32882, #19607, #4939, #34756, #41363, #92031, #25764, #70297, #92494, #83520, #48004, #11095, #47542, #33824, #27186, #76446, #84926, #48957, #13005, #4464, #69333, #33341, #69803, #62238, #26243, #55136, #62734, #42312, #78781, #44162, #65527, #65987, #42780, #13922, #28593, #1098, #36149, #49883, #8197, #37078, #22860, #57027, #57483, #58863, #73068, #6348, #71696, #79258, #71221, #78322, #644, #169, #14399, #29528, #87254, #35221, #21016, #65070, #86324, #28138, #29979, #6825, #92980, #79711, #64147, #35699, #64613, #14853, #43258, #93439, #87710, #13461, #43706, #72156, #85865, #21476, #50354, #86795, #7272, #29048, #57941, #72605, #21954, #50827, #7727, #58408, #36608, #22400, #51272, #80165, #15303, #51726, #52657, #16231, #66431, #80619, #9099, #81537, #23793, #24251, #37976, #16685, #60722, #31373, #89099, #8644, #38911, #82484, #88177, #45540, #73982, #2945, #53125, #15774, #59325, #73535, #82005, #39368, #90039, #30914, #23336, #60262, #88645, #74441, #44633, #17631, #17162, #32298, #9573, #46027, #37521, #38460, #31831, #67366, #74930, #46483, #66884, #10041, #67820, #89561, #1551, #59804, #24731, #30434, #53613, #75386, #10499, #52205, #81087, #2022, #68284, #3406, #61203, #14267, #50698, #40, #65865, #22725, #44960, #30309, #15175, #59197, #7147, #36480, #36022, #51600, #80964, #64939, #16108, #29854, #37400, #21823, #28458, #79586, #87127, #28920, #44033, #66310, #1425, #15636, #57808, #80488, #44505, #65397, #73411, #88045, #73860, #22278, #51150, #35567, #86659, #36952, #43580, #58738, #87581, #79120, #64481, #8521, #23201, #52081, #93308, #14727, #86193, #21345, #72935, #50216, #72478, #7594, #43127, #72032, #510, #29392, #58284, #973, #80034, #8061, #8978, #68507, #11671, #18308, #33442, #62345, #53834, #39128, #91185, #62836, #69907, #91669, #61426, #60945, #48578, #47646, #24958, #54286, #3642, #33927, #68040, #25407, #89794, #26353, #69438, #3166, #54747, #77012, #68981, #32051, #82700, #11205, #32533, #17851, #46702, #90258, #40063, #76074, #76548, #83156, #4111, #19250, #83625, #40520, #75604, #55244, #40986, #10728, #32983, #47165, #84101, #4568, #39584, #61874, #90705, #48108, #26822, #25866, #18787, #12140, #5046, #55709, #84560, #19707, #43357, #21115, #58052, #6451, #71799, #12621, #42410, #28693, #13560, #35326, #72253, #92599, #14025, #49983, #71321, #92134, #56663, #78877, #41467, #57579, #42886, #64252, #49064, #70398, #85034, #78422, #27769, #28236, #56176, #85512, #41941, #6921, #64708, #86903, #7370, #57123, #36251, #77961, #93081, #13103, #93535, #29155, #70853, #22058, #35795, #79364, #63770, #5526, #20658, #85964, #5985, #86424, #14500, #65169, #21579, #34857, #50461, #275, #77478, #34396, #63303, #27289, #20184, #49528, #74095, #16342, #14952, #1663, #23904, #15887, #89215, #50927, #51841, #15408, #65637, #79811, #8303, #80734, #22969, #23450, #37185, #44743, #59916, #30545, #88295, #7827, #38094, #81654, #87358, #73645, #44274, #2140, #52318, #43807, #58513, #72707, #81196, #38576, #36717, #30087, #22508, #59444, #87819, #8755, #750, #16802, #45192, #31488, #37634, #9214, #29634, #66542, #31029, #67004, #88758, #45658, #66093, #52775, #74566, #9695, #51379, #58971, #67479, #80270, #2608, #60376, #73184, #1205, #17283, #31945, #25303, #39478, #68871, #3060, #68398, #82596, #54638, #11561, #33814, #19141, #4001, #47996, #89680, #54181, #24847, #40409, #69795, #53730, #4928, #18670, #26236, #10620, #46140, #3528, #75958, #17743, #32876, #55129, #83994, #4456, #46597, #69327, #33334, #83051, #62231, #76900, #62726, #11089, #39955, #24366, #75496, #25757, #32418, #47536, #76440, #67937, #53244, #91062, #12030, #40877, #82126, #61317, #75043, #10155, #61764, #39022, #90155, #18203, #60836, #47055, #90597, #83512, #42770, #27178, #14393, #57477, #49876, #77367, #84449, #70744, #28585, #42305, #48467, #55601, #71214, #85407, #86318, #13454, #78774, #19599, #6341, #21470, #12503, #5878, #50346, #43252, #20555, #78315, #41355, #57020, #13915, #21009, #84918, #93433, #56065, #92486, #70287, #63193, #41833, #85856, #5420, #92023, #79252, #71689, #72150, #20068, #48949, #34748, #7266, #49425, #77847, #36143, #91556, #26713, #34285, #63663, #12995, #27653, #56552, #35212, #64140, #92973, #28131, #6819, #35693, #64607, #52199, #73976 ),
 ( #639, #30428, #73530, #86789, #37073, #45076, #8639, #65520, #37516, #7719, #81531, #73062, #88170, #51721, #37970, #51267, #14847, #23787, #66426, #163, #74435, #15769, #72599, #1545, #29042, #29523, #65982, #9093, #9566, #1093, #59319, #80611, #23329, #45534, #30908, #29974, #16679, #36603, #81081, #57933, #58403, #58858, #66878, #65062, #87704, #16225, #44628, #2015, #21948, #59798, #22855, #50821, #88639, #87249, #79705, #52651, #43700, #22395, #80160, #44155, #15298, #8192, #89093, #2490, #82929, #32291, #69210, #54058, #90480, #60256, #18081, #4339, #31367, #46476, #33216, #83873, #61196, #25185, #24245, #3881, #25638, #61647, #31825, #40294, #67814, #39362, #53119, #10035, #82478, #32759, #81999, #38905, #62112, #54521, #26107, #2939, #60716, #17625, #55000, #90033, #89555, #90943, #19024, #76781, #17155, #75380, #47878, #38454, #46021, #24723, #68278, #74924, #67360, #83390, #46935, #3400, #18540, #47407, #53607, #10493, #75837, #10960, #39827, #68751, #76317, #11443, #13335, #91439, #41225, #63071, #42176, #41713, #70164, #71567, #6703, #71089, #5756, #28470, #12378, #5299, #20433, #26590, #12875, #34169, #6222, #49301, #33686, #77724, #85744, #78196, #91901, #35091, #48346, #57363, #19947, #64010, #92368, #78658, #27055, #55480, #64492, #92849, #40757, #21356, #56422, #28013, #70629, #55941, #35577, #93318, #56904, #34630, #86205, #84797, #48818, #20891, #84329, #63541, #27529, #49763, #13799, #62595, #85283, #42650, #50226, #11908, #69675, #77249, #4806, #19479, #8532, #65875, #52093, #65409, #28932, #37868, #51612, #14277, #88536, #29865, #86669, #80500, #43138, #79596, #80046, #88056, #23685, #51159, #22738, #984, #73422, #59693, #44971, #15186, #30794, #30320, #14737, #1904, #73872, #37411, #64950, #72042, #58294, #16120, #58750, #36033, #7158, #87592, #72947, #8989, #15648, #66320, #51, #44518, #66773, #57818, #87137, #79130, #21834, #8074, #1435, #50709, #59210, #23213, #80977, #72488, #43592, #7604, #44046, #36492, #519, #29403, #22288, #36962, #53014, #18434, #39719, #40190, #17044, #81891, #2839, #69109, #10391, #24136, #76209, #11338, #90837, #31263, #31721, #33114, #47291, #74330, #45910, #53496, #45429, #52549, #68643, #68171, #82372, #3775, #61548, #9454, #88989, #39256, #60612, #2385, #4234, #74816, #67253, #53958, #38340, #9931, #38805, #16574, #3292, #46372, #83288, #32183, #10856, #60150, #61087, #62002, #67709, #89450, #81425, #24608, #75272, #89928, #17522, #17978, #32660, #75732, #25084, #54417, #82825, #46830, #90381, #25536, #70048, #85178, #83762, #26485, #85640, #13235, #13692, #84227, #55375, #5190, #42544, #77616, #91323, #49660, #78555, #64388, #4697, #34064, #6593, #20788, #47772, #19374, #26951, #18918, #25998, #42071, #41607, #55840, #70986, #34988, #76672, #62483, #12765, #62966, #69569, #71457, #48240, #40650, #27423, #11799, #77142, #12273, #56313, #84695, #41116, #35470, #54883, #20328, #19842, #33574, #91800, #48712, #34529, #70529, #5654, #63437, #49198, #92266, #78093, #6118, #63905, #92740, #27911, #56798, #35927, #16013, #7502, #22632, #79939, #66213, #79495, #43033, #51977, #65771, #28366, #8880, #43937, #7057, #880, #57257, #93672, #406, #8428, #37760, #65300, #36855, #15077, #87482, #73768, #59102, #29294, #44865, #44409, #28830, #93214, #87943, #51504, #79016, #86101, #72385, #30211, #72834, #50119, #14631, #71935, #80866, #29760, #21250, #14169, #7960, #64845, #58640, #57713, #86558, #58189, #37307, #21728, #87031, #80392, #15536, #73316, #50603, #23094, #22183, #43489, #1329, #36387, #51051, #32555, #24980, #52445, #59578, #45793, #3667, #17414, #23578, #30678, #46263, #60504, #61447, #82261, #53854, #88429, #75167, #90278, #81319, #74704, #25429, #18330, #89339, #53375, #16466, #32071, #82719, #89819, #60043, #68530, #2274, #67605, #45320, #38227, #16932, #60968, #74223, #67140, #54307, #17871, #83182, #31157, #88881, #9825, #47186, #24494, #24029, #76098, #11231, #66665, #9342, #38698, #1793, #52905, #81782, #2733, #31613, #10280, #39150, #46723, #68062, #3187, #75626, #10749, #39606, #76569, #26841, #19270, #83647, #86808, #62366, #54770, #41491, #25888, #69458, #91209, #70421, #69928, #4590, #6005, #34880, #5547, #33952, #57953, #40543, #33463, #48599, #18811, #41005, #26377, #34417, #77499, #61895, #12162, #20208, #12646, #55265, #63324, #11692, #21966, #48128, #92155, #55729, #13125, #27312, #47668, #40085, #56198, #180, #63791, #29061, #84120, #90729, #79722, #85057, #77031, #5070, #62856, #50839, #4133, #91689, #84581, #49086, #77984, #33004, #19731, #41961, #70874, #69002, #14864, #15786, #73080, #29540, #43717, #65998, #44645, #80630, #81099, #1110, #73546, #23805, #59337, #52216, #65541, #2035, #45552, #51283, #8655, #8211, #59815, #16242, #72616, #22412, #36619, #45092, #2506, #53137, #87721, #80176, #23348, #51737, #37533, #7738, #74452, #73994, #89110, #66443, #9111, #656, #1562, #88656, #30445, #88189, #9585, #29991, #37987, #66895, #30925, #58420, #22872, #52668, #87266, #81548, #16697, #38473, #15314, #44173, #37089, #67377, #58874, #31384, #60274, #24262, #46496, #18558, #69227, #91456, #76799, #61664, #11925, #53627, #82946, #82497, #4356, #33704, #17645, #62616, #76335, #83890, #68297, #74944, #3418, #39847, #75399, #90496, #19041, #47897, #62129, #10512, #33232, #90960, #18099, #26124, #40774, #26607, #68770, #3899, #82017, #39382, #83406, #90050, #11461, #69692, #32313, #38924, #17175, #25655, #2958, #61216, #25203, #4821, #46039, #54076, #67833, #40312, #47425, #10054, #32776, #55020, #46953, #31844, #60733, #75855, #10977, #89573, #24745, #54538, #85301, #27545, #28030, #12892, #20450, #64507, #6238, #92867, #12395, #42666, #86219, #91917, #49317, #19962, #6719, #56919, #84347, #63089, #77266, #85758, #43154, #66, #34646, #27072, #64026, #92385, #56437, #48362, #21370, #20908, #36047, #78212, #49777, #19496, #13351, #35592, #42192, #71104, #50240, #70644, #78672, #13814, #35107, #70183, #63557, #71582, #41241, #93333, #28484, #57378, #55958, #5317, #84812, #79145, #5772, #14294, #34185, #72056, #48835, #7173, #64965, #55498, #77741, #41730, #23697, #534, #29880, #29419, #44984, #74344, #58309, #9468, #23226, #30808, #15200, #21850, #44060, #80513, #87152, #8545, #59707, #88550, #9002, #22302, #73885, #37880, #58764, #66786, #52561, #67267, #15664, #44532, #28946, #51173, #30333, #36977, #52107, #80990, #72502, #57832, #16132, #81440, #16588, #80060, #1916, #45443, #87606, #38353, #86684, #50725, #73435, #37425, #79610, #72961, #59224, #65889, #14751, #43606, #7620, #36507, #65422, #8089, #1001, #22752, #51627, #66335, #1448, #88070, #17058, #46387, #89464, #26017, #60163, #17536, #53028, #25551, #61561, #89002, #46846, #69123, #61103, #40667, #2398, #3308, #60626, #45923, #31278, #53510, #32197, #68187, #68656, #82388, #89942, #11354, #75747, #39733, #81905, #83303, #33129, #38818, #25099, #24625, #47308, #3792, #24149, #9946, #74833, #32674, #83778, #67724, #75286, #2853, #10870, #39270, #53972, #31735, #62018, #90393, #76690, #82840, #54430, #10406, #17992, #76223, #18449, #40207, #90852, #4250, #54900, #18933, #47788, #11815, #48730, #42085, #4714, #49673, #13250, #92282, #41134, #62501, #77159, #70545, #84712, #20343, #48257, #19860, #34081, #6133 ),
 ( #77634, #92758, #27925, #19393, #69585, #56814, #28381, #35488, #57273, #26968, #26501, #14187, #71002, #84243, #12783, #62984, #93229, #33592, #41625, #55392, #85655, #35004, #91339, #49213, #42559, #34543, #12289, #70066, #5668, #91816, #5208, #55859, #63451, #27438, #56331, #63920, #85194, #78110, #78569, #20804, #13707, #71476, #6608, #64402, #86116, #21265, #50136, #79035, #44428, #71952, #50621, #64860, #15557, #30699, #81337, #22200, #79511, #51523, #79956, #15095, #35943, #8900, #80409, #23596, #65788, #37324, #7071, #7979, #87962, #72852, #897, #37778, #58206, #73334, #8445, #36873, #57729, #51070, #66232, #93688, #23114, #1346, #29780, #14649, #28845, #43505, #43954, #87051, #87502, #21745, #58659, #7519, #30230, #59120, #52463, #66685, #22650, #1811, #72402, #51998, #36405, #80884, #88448, #65318, #43048, #16032, #44883, #29312, #86576, #73785, #59597, #425, #10299, #68550, #3688, #75644, #16949, #17889, #10767, #89357, #39625, #61466, #47203, #17432, #75185, #16484, #45340, #24513, #74722, #31176, #74241, #67623, #82281, #53395, #89838, #2750, #46282, #32573, #68080, #60991, #60061, #46742, #90296, #81802, #39168, #9843, #25448, #25000, #38246, #52923, #2292, #53871, #18348, #9362, #3205, #45815, #82737, #32089, #54325, #88899, #83201, #67160, #24048, #38715, #31630, #60521, #66077, #52303, #37169, #58955, #2124, #22491, #37617, #73629, #1189, #22042, #80255, #8740, #36236, #81180, #44728, #30070, #72692, #257, #14937, #8288, #51364, #51826, #79795, #15391, #65622, #66528, #88280, #16785, #31013, #80719, #59900, #7811, #87803, #36701, #23435, #52757, #734, #81638, #1647, #9197, #87342, #29140, #44258, #22952, #29619, #15872, #38075, #66986, #16326, #58497, #45176, #74078, #30527, #88742, #23888, #45639, #59429, #7354, #65154, #73169, #58036, #86888, #50911, #43792, #24350, #74548, #61749, #33320, #40394, #62217, #31928, #31472, #19127, #18188, #89198, #24831, #67920, #4440, #38561, #89662, #60360, #3985, #39940, #67463, #25288, #47520, #39464, #9679, #26220, #10140, #55114, #68856, #76425, #60819, #2592, #53714, #32404, #39006, #54166, #11547, #69312, #54623, #3044, #25742, #83495, #10606, #18653, #91046, #53225, #61302, #90138, #82107, #82581, #75941, #17728, #32860, #90581, #17266, #46124, #83979, #75027, #46583, #75481, #68381, #3512, #83035, #47040, #11071, #92009, #41339, #71670, #12013, #63178, #4912, #71198, #13439, #40863, #92470, #20993, #12980, #86302, #47982, #77832, #12487, #62712, #69781, #5406, #41818, #70729, #49410, #34271, #5862, #57004, #27636, #85392, #33798, #35193, #78758, #84435, #34732, #70273, #92957, #78300, #91542, #55587, #26698, #42286, #35677, #19583, #27161, #48452, #56535, #84903, #63648, #77353, #13899, #6325, #28569, #64121, #28116, #56049, #85841, #49859, #42753, #6804, #64592, #93417, #57459, #87687, #15281, #36126, #620, #22840, #50327, #1528, #58844, #44138, #86770, #14376, #29026, #22378, #36587, #65967, #146, #65501, #79688, #51707, #8625, #30891, #16211, #1078, #45062, #21931, #51251, #50803, #37502, #73043, #14830, #29958, #52185, #81066, #30414, #43684, #66411, #59305, #80141, #88153, #73962, #59784, #8173, #37057, #21454, #72580, #80595, #29505, #44612, #73516, #65043, #79234, #23312, #9076, #37956, #66863, #7702, #72134, #43236, #15752, #57913, #58387, #87230, #1998, #7250, #10021, #45519, #18070, #54046, #52637, #39346, #61636, #53592, #33205, #88625, #89543, #53105, #9550, #23772, #46005, #24706, #60703, #61181, #74910, #82465, #3869, #68265, #32275, #74421, #75825, #25626, #31353, #17612, #81983, #39815, #90019, #81517, #2476, #16664, #25172, #76305, #38437, #67800, #60241, #3387, #31810, #46463, #67346, #54508, #82916, #69199, #75366, #46923, #89079, #10480, #68738, #10949, #32748, #83380, #38891, #90469, #18528, #47394, #24228, #2925, #11431, #17139, #40282, #4328, #84785, #33673, #54984, #69662, #63059, #77235, #12862, #40745, #12365, #26578, #92357, #49290, #71557, #56894, #41701, #85733, #62582, #91888, #91424, #78185, #13788, #55467, #42640, #56412, #64000, #48334, #83860, #41213, #19935, #20879, #70150, #27518, #34620, #55930, #76768, #5286, #63530, #90930, #42164, #5745, #48805, #84316, #19013, #4794, #27042, #34156, #70618, #19467, #77712, #85272, #20421, #13323, #6692, #49751, #71080, #78648, #6212, #35081, #92838, #28001, #62097, #26095, #47865, #11896, #48317, #32731, #39329, #61619, #4310, #75806, #26077, #77218, #12346, #26561, #39798, #91406, #55450, #76287, #84301, #41195, #84767, #33188, #62078, #46446, #10930, #47848, #54491, #69646, #4774, #90001, #75348, #33656, #5269, #70133, #34138, #3850, #3371, #10463, #83842, #61164, #90451, #68720, #63041, #68247, #25608, #32259, #62565, #11878, #25156, #90911, #19451, #11413, #54030, #82897, #47373, #83359, #18053, #46905, #18509, #40264, #69181, #18995, #54966, #76750, #91872, #40729, #27026, #55915, #7132, #50682, #56394, #78630, #78169, #64921, #21327, #48788, #27496, #41683, #86176, #7579, #58269, #92822, #85256, #28441, #56876, #85717, #12845, #79568, #57334, #491, #42621, #14250, #77696, #13772, #24, #49733, #13307, #50197, #27985, #43108, #72015, #63513, #70601, #36003, #72460, #14711, #36464, #71063, #5728, #34603, #79101, #92341, #63982, #42145, #43564, #20404, #35062, #49274, #28903, #57791, #6195, #64463, #86641, #71540, #20862, #6673, #35550, #93290, #65379, #29375, #44489, #23180, #59179, #59663, #73393, #52063, #2355, #37837, #30761, #44017, #74298, #24105, #29836, #80945, #51582, #38309, #88506, #22261, #957, #15158, #23653, #74784, #31687, #66292, #58719, #1869, #30291, #88023, #80018, #52986, #52519, #67679, #16090, #81395, #51135, #44942, #67224, #73842, #8958, #81860, #8503, #16543, #45399, #66743, #8041, #1404, #9422, #72914, #31233, #60119, #88958, #87563, #36935, #22708, #17009, #37382, #45878, #65849, #9901, #80468, #38775, #2805, #87111, #15617, #40159, #55342, #32151, #61517, #61052, #76640, #12236, #89895, #41083, #54845, #62444, #46797, #53459, #75699, #18402, #25053, #69076, #91287, #26453, #40617, #53926, #11765, #69533, #90348, #4666, #84193, #5150, #47261, #76175, #60582, #82794, #82340, #68140, #25504, #10824, #11307, #39222, #39684, #17946, #90805, #47742, #70007, #19341, #4204, #48203, #68608, #54382, #3745, #33539, #89417, #32627, #24571, #83727, #77105, #83258, #17488, #33079, #61968, #25964, #18887, #46340, #75242, #10357, #3261, #78977, #42994, #63868, #14129, #28790, #72347, #85606, #49624, #34027, #92231, #35432, #42036, #57222, #86062, #77577, #62931, #21212, #86520, #93633, #21685, #85136, #84656, #91765, #71421, #48676, #78058, #27387, #57677, #26917, #49165, #19808, #50082, #93180, #55804, #78520, #7020, #92702, #12728, #41571, #34956, #56277, #70493, #5621, #20291, #27872, #6082, #6553, #13200, #56765, #71900, #13657, #64354, #34496, #35891, #64809, #63402, #20753, #70950, #50562, #28332, #42509, #79459, #14593, #43450, #88847, #45756, #80358, #15041, #15979, #44370, #73281, #368, #67103, #44831, #81748, #30177, #1755, #36348, #66178, #52412, #37272, #59061, #2237, #22594, #37724, #73734, #1295, #22148, #15499, #8846, #65262, #81287, #66630, #87909, #23060, #51938, #7465, #65734, #30642, #8394, #59541, #88391, #51016, #29254, #23542, #60007, #31121, #23996, #58607, #58150 ),
 ( #16433, #845, #9307, #36813, #80828, #86996, #72798, #51469, #45285, #79903, #7922, #52869, #74188, #16898, #29726, #87448, #38189, #43901, #32515, #46230, #4553, #33427, #19235, #53339, #24941, #55230, #40503, #2698, #68026, #75590, #67569, #74666, #61860, #90243, #10713, #90691, #83611, #31580, #17378, #61411, #53818, #24460, #26337, #3153, #89304, #76060, #60469, #10244, #32036, #11189, #39570, #39113, #69422, #62331, #40049, #68492, #91171, #75134, #60931, #83142, #82224, #3627, #89778, #68966, #18293, #82686, #46688, #54733, #47151, #17836, #4096, #25392, #84085, #54272, #32967, #25851, #47630, #18772, #76534, #9790, #11656, #38665, #57566, #92585, #55694, #49516, #12125, #40971, #84545, #49050, #63287, #27754, #26808, #92120, #12607, #78408, #35312, #86409, #42872, #56650, #71785, #19692, #77945, #48561, #64237, #93521, #77464, #28680, #42396, #49970, #34382, #69893, #27274, #5971, #41452, #85499, #78862, #14012, #28222, #70384, #93068, #57110, #13089, #85950, #6907, #48092, #34844, #63755, #76996, #5512, #13547, #56161, #71307, #6437, #91655, #5032, #21102, #35782, #64695, #33912, #85018, #62821, #20170, #20646, #41927, #70838, #14938, #45177, #79350, #36702, #72240, #44729, #80720, #14485, #66078, #88281, #80256, #59901, #21565, #22492, #79796, #36237, #50448, #72693, #51365, #87343, #87804, #7812, #15392, #30528, #1190, #58956, #7355, #8741, #52304, #58037, #44259, #43793, #66529, #22953, #43343, #29141, #65155, #51827, #9198, #258, #735, #86889, #30071, #58498, #73170, #22043, #81181, #15873, #2125, #8289, #73630, #50912, #37170, #1648, #37618, #59430, #16327, #65623, #23436, #74079, #38076, #29620, #66987, #31014, #23889, #68857, #32405, #17729, #60361, #75942, #18189, #82108, #90582, #24351, #89663, #16786, #89199, #39007, #54167, #52758, #53226, #54624, #11072, #76426, #17267, #46125, #67921, #11548, #46584, #75028, #18654, #47521, #33321, #67464, #3045, #69313, #83496, #45640, #10141, #24832, #81639, #88743, #39941, #10607, #53715, #3986, #32861, #74549, #31473, #75482, #31929, #38562, #40395, #60820, #9680, #90139, #2593, #82582, #39465, #25289, #68382, #3513, #4441, #61303, #83036, #47041, #61750, #25743, #91543, #70730, #47983, #63179, #26699, #27637, #5863, #83980, #34272, #42287, #34733, #62713, #63649, #4913, #78759, #70274, #85393, #48933, #35194, #48453, #12014, #20994, #92471, #91047, #71671, #12981, #69782, #56536, #26221, #55588, #92010, #71199, #6805, #27162, #20541, #77833, #49411, #42754, #28117, #56050, #13900, #13440, #84436, #62218, #57005, #78301, #76886, #55115, #41340, #92958, #41819, #19128, #40864, #6326, #84904, #85842, #64122, #49860, #33799, #19584, #77354, #12488, #5407, #20052, #82355, #30779, #23669, #93418, #2370, #7251, #79689, #31248, #28570, #36127, #2822, #24122, #24589, #147, #65044, #14831, #53478, #88521, #29027, #60597, #89432, #75257, #14377, #43685, #17503, #31704, #57460, #57914, #37854, #86303, #35678, #53001, #52535, #66758, #81875, #45895, #21455, #72135, #81410, #72581, #79235, #46356, #86771, #50328, #38326, #43237, #21932, #50804, #67240, #1887, #7703, #64593, #59678, #60135, #16560, #45414, #74315, #9439, #88974, #17029, #74800, #9917, #38790, #67694, #32167, #76191, #84207, #18900, #10837, #76653, #46812, #26929, #18415, #33552, #90818, #77120, #90362, #53939, #62944, #11780, #39239, #19822, #54862, #17959, #40630, #68155, #39700, #11321, #19354, #48688, #40172, #47755, #25977, #4678, #84673, #70023, #69091, #55817, #55355, #68624, #10372, #5166, #62461, #89911, #3275, #83271, #41095, #83743, #61068, #25067, #69548, #4217, #34041, #91303, #26466, #82808, #48218, #91778, #75714, #47275, #3758, #32643, #33092, #12249, #61531, #25519, #54398, #61983, #70964, #79474, #13214, #78533, #5634, #43466, #35905, #63416, #70507, #56778, #14608, #28345, #34509, #41585, #57235, #71434, #72363, #93193, #64823, #92245, #86077, #7480, #27402, #85620, #36365, #29271, #6570, #64367, #56290, #43010, #93647, #7035, #6096, #65278, #42050, #13672, #85153, #49177, #27888, #71914, #20306, #78071, #383, #28807, #58167, #34968, #63882, #20766, #87011, #35448, #92718, #22163, #77593, #12743, #49638, #42522, #21228, #50097, #78991, #14146, #57691, #86534, #21702, #50579, #66647, #80846, #38205, #60024, #43918, #87463, #37739, #30192, #860, #2713, #73297, #65751, #52427, #36832, #80373, #8409, #81302, #15994, #15514, #16913, #45771, #16448, #44846, #67584, #51485, #44388, #59558, #29741, #51954, #37287, #45300, #88408, #72813, #23075, #31137, #23559, #66194, #74205, #22610, #31594, #59081, #9322, #1773, #24010, #1310, #58622, #9805, #67119, #79919, #60483, #30657, #87924, #2254, #15056, #73749, #8861, #88861, #89320, #52883, #81763, #74681, #38679, #51031, #7939, #54287, #69908, #69439, #53835, #40987, #68982, #18310, #55245, #40064, #76549, #46244, #4112, #84102, #82239, #32534, #19251, #5047, #47166, #11206, #17395, #83626, #11672, #47647, #17852, #26354, #82701, #25408, #75148, #89795, #68508, #18788, #10260, #24959, #48109, #40521, #12141, #46703, #75606, #3643, #33929, #76075, #10729, #77013, #62837, #24475, #3167, #61427, #53354, #39130, #68041, #39585, #83157, #32052, #60946, #4569, #32984, #61875, #33443, #62346, #90259, #90706, #25867, #54749, #91187, #43358, #20185, #12622, #93082, #77479, #27290, #49065, #28237, #27770, #56177, #57580, #86425, #57124, #85513, #14501, #92135, #85035, #6452, #41468, #92600, #77962, #85966, #35327, #19708, #63771, #71800, #64253, #13105, #21116, #34397, #72254, #5986, #49984, #78423, #64709, #41942, #70400, #50462, #78878, #26823, #7371, #42411, #5527, #14026, #55710, #70854, #56664, #6922, #36252, #20659, #42887, #13561, #35796, #91670, #21580, #49530, #84561, #93536, #34858, #48579, #79365, #28695, #63304, #71322, #44276, #2141, #15888, #22059, #29156, #23905, #31030, #52776, #22509, #50928, #9696, #8756, #79812, #15409, #58514, #88759, #58053, #80271, #14953, #88296, #30546, #86904, #44744, #38095, #30088, #65171, #276, #66094, #29635, #43808, #72708, #51380, #1206, #37186, #37635, #73185, #58972, #74096, #73646, #66543, #7829, #52319, #59918, #36718, #87820, #87359, #16343, #1664, #65638, #751, #8304, #59445, #81655, #22970, #51842, #80736, #23452, #81197, #45193, #9215, #16803, #67005, #45659, #74567, #32877, #67480, #3529, #83514, #68400, #90156, #33335, #53731, #68872, #11090, #32419, #53245, #17744, #39956, #2610, #18671, #75960, #61318, #10156, #31489, #46141, #39479, #82597, #83052, #17284, #46598, #3061, #4002, #25758, #47997, #62232, #18205, #91065, #39024, #25304, #67938, #54640, #83995, #31946, #19142, #61765, #40410, #24848, #60377, #75498, #54182, #60838, #47056, #69328, #4458, #47537, #89681, #76441, #11562, #90598, #26237, #55130, #76901, #38577, #89216, #24367, #10621, #82127, #75044, #35214, #64141, #55602, #12031, #92974, #63664, #27655, #40878, #70289, #13455, #20070, #28132, #57021, #84450, #69796, #85858, #64608, #71690, #93434, #63194, #62727, #50348, #49427, #26714, #56066, #5421, #35694, #4930, #27179, #91557, #21010, #71215, #33816, #56554, #78775, #70745, #19600, #48468, #12997, #34286, #77368, #12505, #92024, #41834, #77848, #78316, #84919, #5879, #49877, #85408, #42306, #41356, #13916, #42772, #48950, #34749, #92487, #6820, #6342, #20556 ),
 ( #28587, #57478, #86319, #21471, #14394, #59320, #22856, #8193, #50822, #72151, #86790, #80161, #640, #29975, #57935, #29524, #43701, #15770, #66427, #88640, #73977, #58859, #9094, #79706, #15299, #14848, #1546, #30909, #72600, #59799, #73531, #81082, #65522, #7267, #58404, #37074, #7721, #87705, #16226, #45077, #88171, #36604, #30429, #23331, #44157, #52200, #37971, #23788, #51722, #66879, #43253, #87250, #2016, #79253, #73063, #65983, #36144, #44629, #65064, #8640, #22396, #164, #51268, #1094, #29043, #80613, #37517, #21949, #16680, #53120, #18541, #39828, #40295, #17156, #82000, #2940, #69211, #10494, #24246, #76318, #11444, #90944, #31368, #31826, #33217, #47408, #74436, #46022, #53608, #45535, #52652, #68752, #68279, #82479, #3882, #61648, #9567, #89094, #39363, #60717, #2491, #4340, #74925, #67361, #54059, #38455, #10036, #38906, #82930, #17626, #67815, #62113, #81532, #18082, #46477, #60257, #89556, #24724, #61197, #75381, #3401, #32292, #46936, #90034, #25186, #75838, #32760, #10961, #90481, #25639, #54522, #83391, #34170, #49302, #12876, #92850, #12379, #69676, #78659, #92369, #55001, #35578, #70630, #33687, #27530, #83874, #26591, #27056, #35092, #64493, #91902, #63542, #41714, #20434, #6704, #85745, #55942, #71568, #71090, #55481, #42651, #20892, #78197, #11909, #19025, #5300, #56905, #5757, #76782, #47879, #34631, #19948, #49764, #56423, #13336, #40758, #42177, #26108, #13800, #84798, #4807, #6223, #84330, #62596, #91440, #64011, #19480, #48347, #63072, #77250, #85284, #41226, #70165, #28014, #48819, #77725, #58296, #36964, #21357, #87139, #51614, #28471, #79598, #80502, #66322, #36494, #29405, #57364, #44048, #65877, #8076, #28934, #15650, #64952, #43594, #86206, #7160, #50711, #72949, #50227, #36035, #44520, #986, #73424, #53, #57820, #21836, #37413, #521, #86671, #8534, #1437, #30322, #43140, #14739, #93319, #79131, #72490, #7606, #22290, #72044, #14278, #65411, #51161, #80048, #15188, #29867, #22740, #58752, #87594, #63389, #34015, #35877, #12715, #5136, #85592, #69996, #19796, #41557, #20739, #20275, #48665, #50067, #78963, #49610, #78046, #7005, #84645, #77566, #92688, #62918, #85124, #70480, #78505, #27858, #12224, #56264, #64338, #56749, #5608, #13643, #26905, #64794, #92219, #42494, #70937, #57206, #34483, #91753, #42977, #71408, #19330, #93618, #34941, #55793, #6540, #48192, #27374, #49150, #93165, #28776, #13187, #35417, #6068, #42022, #28317, #84182, #63855, #77094, #86047, #21196, #14114, #41071, #71883, #15487, #86982, #37260, #88377, #23527, #37711, #51003, #8833, #66617, #87436, #1740, #52396, #2222, #44358, #73268, #57660, #22135, #59047, #65719, #80815, #15964, #7452, #86507, #44818, #16419, #81273, #45271, #15029, #14580, #21670, #1282, #72333, #7909, #79890, #74174, #50547, #72784, #43437, #73721, #23047, #79444, #8380, #30627, #22582, #36334, #65248, #58595, #43888, #354, #29241, #36799, #51456, #29713, #30164, #831, #80345, #59528, #66166, #87894, #58136, #9291, #38174, #51925, #67089, #89290, #77335, #33777, #59993, #38651, #52855, #4893, #20034, #70712, #10229, #67555, #40843, #68009, #3138, #23982, #91990, #69762, #12962, #53802, #26679, #88832, #89763, #12469, #60917, #82670, #27143, #46215, #62690, #91523, #24925, #45740, #39097, #55569, #81733, #41316, #84417, #17818, #2684, #16881, #31564, #32018, #75119, #75575, #9776, #46672, #24443, #19565, #48431, #41801, #56028, #11994, #84883, #60455, #70253, #63159, #5388, #34253, #74651, #48911, #77813, #53324, #31106, #82209, #17364, #93400, #86284, #63629, #65029, #86753, #29012, #92938, #7687, #35176, #6783, #27617, #71179, #49842, #129, #92454, #6308, #65487, #21915, #87214, #64098, #28099, #78739, #22362, #57443, #56986, #29487, #58372, #44122, #78283, #13882, #80124, #604, #56514, #85824, #35660, #85373, #5843, #50789, #21437, #64575, #79674, #14815, #20523, #42266, #50311, #42735, #49391, #51236, #20975, #13421, #7236, #71650, #28552, #79216, #36111, #14359, #43219, #15263, #34715, #57897, #72120, #43670, #72565, #36572, #81501, #58826, #73945, #8609, #38419, #16648, #1062, #45044, #53087, #45502, #73497, #74404, #15732, #89526, #81049, #2460, #59767, #45988, #59289, #22821, #31792, #9534, #8154, #82448, #23756, #80579, #67328, #37037, #37485, #9060, #81966, #17596, #37938, #31336, #88608, #60223, #53573, #38875, #66847, #24689, #24212, #66395, #73026, #67782, #89062, #87671, #65951, #52166, #10004, #52619, #29941, #51690, #17122, #1982, #1511, #74893, #44593, #30397, #88135, #2908, #60686, #23293, #16192, #30873, #87356, #65167, #15406, #1661, #30542, #15885, #29153, #80732, #44741, #65634, #73643, #59442, #74092, #22506, #51377, #35793, #273, #37183, #43805, #58969, #87816, #79362, #64706, #22967, #88293, #23448, #52316, #86901, #86422, #93533, #73182, #50459, #79809, #58050, #81193, #28691, #50925, #21577, #51839, #1203, #57577, #80268, #8753, #748, #14497, #43355, #36714, #22056, #72251, #7368, #14950, #29632, #7825, #8301, #72705, #58511, #37632, #44272, #66090, #36249, #16339, #45189, #30085, #67934, #67476, #54178, #10617, #38091, #16799, #31026, #75493, #90594, #47533, #82123, #45655, #17740, #46137, #75040, #2137, #68868, #46594, #83509, #31942, #3525, #67001, #3057, #83048, #39019, #60833, #3998, #24363, #39475, #68395, #89677, #23901, #17280, #32415, #59913, #18200, #61314, #24844, #74563, #88755, #9692, #10152, #53241, #53727, #81651, #82593, #2605, #90152, #25300, #18667, #32873, #47052, #61761, #38573, #75955, #11086, #25754, #31485, #60373, #39952, #54635, #9211, #89212, #52772, #6337, #21005, #55126, #26710, #57016, #42300, #4452, #69792, #77364, #69324, #76437, #63659, #92020, #12500, #92482, #85403, #33331, #19138, #63190, #55598, #26233, #28127, #4925, #91059, #77843, #62228, #12026, #33811, #12991, #41352, #40874, #71210, #35208, #41829, #70284, #92969, #76897, #62723, #84914, #83991, #5417, #91553, #70740, #20064, #47993, #48464, #56548, #48945, #84446, #5874, #19595, #85852, #34282, #34743, #27173, #49421, #56061, #27649, #64136, #20551, #11558, #40406, #78311, #13450, #51263, #13911, #50342, #50817, #58855, #59316, #21944, #87245, #65516, #44151, #30425, #15766, #79701, #1541, #1089, #79248, #66423, #44625, #8188, #35689, #42766, #29038, #80608, #635, #6815, #71685, #29519, #43696, #73527, #58399, #37069, #64603, #22391, #8636, #93429, #57929, #37513, #88167, #72594, #36599, #28581, #15294, #65978, #73058, #43248, #51718, #14389, #14843, #57472, #21466, #159, #29970, #86314, #72146, #49871, #7262, #86785, #78770, #80155, #36139, #65057, #87700, #7715, #22852, #38902, #75377, #45073, #2936, #54056, #81078, #31364, #82926, #68749, #17152, #10032, #16222, #82475, #10490, #46473, #16675, #25182, #52648, #24241, #73973, #88636, #67357, #17622, #9089, #23784, #18079, #39358, #10958, #81528, #45531, #2487, #39825, #74921, #74432, #46932, #75835, #61645, #2012, #60253, #3879, #32757, #37967, #9563, #53116, #66875, #23326, #68275, #67811, #81996, #3397, #32288, #30905, #59795, #31821, #89090, #38451, #52196, #46018, #60713, #24720, #89552, #53604, #61193, #90030, #26588, #54998, #57702, #86545, #57246, #84327, #14620, #90941, #26105, #5297, #76315, #91436, #83870, #86088, #34167, #18538, #62593, #71925, #63069, #19022, #91899 ),
 ( #79003, #50591, #21716, #79485, #47876, #47405, #36376, #27053, #55478, #19477, #21239, #76779, #48344, #7046, #41223, #50108, #11441, #14158, #28818, #33214, #77246, #11906, #43022, #35916, #25635, #4337, #40292, #64834, #43477, #90478, #69672, #62109, #93658, #33684, #12376, #83388, #72374, #7491, #54518, #70162, #69208, #40755, #4804, #16456, #1319, #23084, #60033, #80382, #1782, #37748, #59091, #79928, #44398, #66656, #394, #45308, #8870, #87933, #36844, #58180, #72823, #66203, #15523, #16003, #43927, #73307, #29750, #30666, #52435, #74692, #88870, #44855, #24019, #65761, #30201, #871, #81310, #16922, #58631, #45781, #59569, #67129, #51494, #87022, #8418, #51964, #87472, #73758, #2264, #31146, #74213, #22619, #9332, #38215, #80856, #52893, #81772, #9815, #88418, #23568, #65289, #37297, #29284, #22173, #51041, #15065, #7948, #38688, #25877, #91197, #4578, #26365, #89807, #89329, #77021, #76086, #53364, #82710, #32061, #62355, #2723, #53844, #24484, #61885, #4122, #31603, #83169, #11682, #3655, #67594, #60492, #39596, #3177, #82250, #17405, #24969, #46253, #68519, #60956, #75157, #10269, #17861, #32545, #10739, #11219, #46712, #61437, #47658, #18320, #40075, #39139, #54759, #69448, #68050, #90268, #75615, #83636, #68992, #25419, #54297, #47176, #32994, #55255, #90717, #18799, #76559, #40532, #33453, #84110, #19260, #48118, #49540, #86433, #34868, #6463, #40995, #70864, #57134, #41951, #63781, #6932, #27300, #42421, #78435, #5995, #26831, #85047, #13571, #69918, #85976, #71333, #92610, #77489, #5057, #19718, #13115, #56187, #56674, #84571, #20196, #70411, #35338, #93093, #21592, #35805, #85523, #64719, #12634, #27781, #41479, #28247, #57589, #5536, #50471, #64263, #14036, #92145, #33940, #49074, #20668, #34407, #21126, #42898, #71810, #49994, #63314, #78889, #93545, #28704, #12150, #62846, #91680, #55719, #48589, #77973, #43817, #80745, #87367, #8764, #37643, #29165, #79374, #66551, #38104, #45201, #67014, #36726, #36261, #23914, #22979, #285, #29644, #72716, #9223, #43367, #759, #65182, #1673, #44753, #72263, #30096, #52328, #44286, #14511, #22068, #66102, #58524, #58061, #31039, #7839, #86913, #15896, #50936, #14961, #65645, #73654, #15418, #22517, #74104, #2149, #30555, #73193, #59929, #79820, #51388, #87828, #80279, #8312, #37195, #59453, #51853, #7381, #1214, #88304, #23461, #58980, #81205, #16351, #88768, #60848, #75973, #39489, #25770, #39034, #2620, #11573, #25315, #81664, #62244, #3541, #60386, #54194, #16812, #53255, #53741, #61776, #91079, #24857, #90167, #68412, #47067, #33347, #18684, #82607, #4470, #4013, #82137, #69339, #47548, #11102, #38586, #45669, #31955, #83526, #32430, #9705, #74577, #61329, #46607, #76452, #83063, #39967, #67489, #18217, #40421, #31498, #89691, #52786, #89225, #75509, #68883, #24376, #32889, #90609, #54652, #46150, #17294, #75054, #17754, #10165, #67947, #3070, #10631, #84006, #26728, #85871, #13468, #13928, #84463, #55614, #70303, #42786, #77861, #91571, #49890, #78787, #64619, #4945, #5434, #6831, #21022, #48010, #19613, #27192, #19154, #26250, #42318, #41847, #56079, #71227, #35227, #76914, #5892, #71703, #48482, #84932, #77381, #6354, #35705, #12519, #55143, #20568, #28144, #41369, #12044, #34300, #13011, #63207, #34762, #57033, #40891, #64153, #92037, #92986, #69809, #20084, #33831, #62740, #48965, #70759, #63677, #92500, #27669, #56567, #85420, #49440, #78328, #43264, #93445, #80626, #52212, #59333, #81094, #50834, #50360, #37983, #37085, #14405, #43713, #86803, #23344, #57489, #14860, #79265, #22868, #58870, #86331, #44169, #66438, #58415, #28599, #21482, #652, #57948, #72162, #7278, #79718, #29535, #65535, #65994, #72612, #87261, #8651, #73075, #1105, #36155, #15782, #30441, #65077, #22407, #21961, #44640, #29986, #176, #29056, #7734, #87717, #16238, #36615, #51279, #80172, #8206, #15310, #51733, #73542, #88184, #37528, #73989, #1558, #45088, #9106, #31839, #18093, #2953, #24738, #61659, #82012, #3412, #39375, #60729, #81544, #46034, #68291, #2030, #46947, #10506, #89568, #38469, #59811, #74448, #67828, #17169, #17639, #45547, #74939, #31380, #32305, #54071, #76330, #90491, #23800, #82941, #3894, #9580, #53621, #60269, #75849, #61210, #30921, #67373, #88652, #90045, #54533, #11455, #10049, #2502, #75393, #38919, #82491, #52664, #32771, #25197, #47420, #46490, #10972, #16692, #39840, #68764, #25650, #83402, #18552, #66891, #89106, #24258, #53132, #55013, #19492, #12888, #69222, #20446, #77737, #63084, #11920, #33228, #47891, #41237, #55493, #84809, #19036, #84341, #4817, #70641, #27541, #49774, #35104, #19959, #64022, #40769, #70177, #69687, #56433, #85755, #33698, #20902, #34643, #42188, #26602, #62124, #48358, #91913, #62609, #48830, #71101, #6234, #49314, #91452, #85296, #78208, #5312, #13347, #92862, #78669, #27067, #55954, #40307, #77261, #41725, #12391, #63553, #92382, #83886, #4351, #28026, #56915, #90955, #26119, #34181, #76794, #5769, #51169, #28480, #57829, #7169, #37421, #71579, #28943, #64503, #36972, #72956, #6715, #58305, #80510, #72498, #52102, #13810, #14747, #72053, #57373, #42662, #64961, #43602, #79606, #80056, #62, #7615, #22748, #87148, #15196, #36044, #43150, #86679, #30330, #65418, #79140, #66332, #1445, #35589, #86215, #21844, #88065, #73432, #93329, #50721, #36502, #21367, #50237, #995, #29414, #529, #29876, #51623, #14289, #22298, #44056, #8084, #65886, #59220, #58760, #87602, #15658, #44528, #8542, #23222, #82381, #17054, #45439, #46839, #75742, #46381, #74827, #3786, #81435, #16583, #89459, #66783, #81901, #74340, #75281, #24620, #8999, #53023, #61098, #53505, #9464, #17531, #23694, #32670, #88998, #10400, #67718, #53967, #67262, #30803, #39728, #39265, #16129, #90389, #31730, #88546, #68181, #44980, #38349, #45919, #89937, #25545, #9941, #3302, #2849, #32193, #61556, #10865, #38814, #80987, #25093, #2395, #73881, #68651, #82834, #1913, #37877, #60159, #17987, #60621, #59702, #52558, #31272, #24145, #85190, #70062, #12778, #76218, #34077, #20338, #18445, #62496, #49208, #6129, #48252, #41129, #47303, #19855, #41620, #77628, #47784, #56326, #83773, #55388, #11348, #26010, #4709, #48726, #40202, #54896, #78104, #70541, #42081, #33124, #69581, #18929, #84708, #5663, #63916, #13245, #62979, #70997, #76685, #84239, #11810, #34539, #35000, #40661, #92753, #63447, #54426, #33587, #69118, #91335, #12285, #26497, #91812, #83297, #4244, #92278, #19389, #27434, #62013, #77154, #90848, #5203, #26964, #55855, #43502, #27921, #86112, #29309, #35939, #51065, #79952, #71472, #56809, #15090, #80405, #87497, #15552, #79030, #78565, #66228, #65315, #42555, #71948, #21261, #51518, #85651, #43045, #13703, #43950, #87047, #20799, #72398, #893, #86573, #49669, #6604, #28842, #50131, #35482, #64398, #14184, #57726, #93684, #422, #7068, #21742, #36869, #7516, #58203, #93224, #72847, #58655, #28377, #50618, #64857, #7975, #22196, #57268, #79508, #14645, #65784, #44424, #36401, #29776, #22646, #73330, #8441, #37320, #87957, #62262, #39984, #76932, #24044, #90625, #30225, #60057, #47564, #31171, #52919, #91095, #16480, #32905, #68900, #88895, #16028, #74237, #4032, #59116, #76469, #61793, #81798, #66680, #23110, #8896, #2288, #45336, #47084, #23592, #44879, #25787, #80881, #30693, #52459 ),
 ( #54668, #18233, #69355, #81333, #73781, #55160, #83542, #51993, #12060, #75989, #37774, #18700, #1807, #59593, #11118, #11590, #40907, #67155, #40438, #4485, #33362, #1342, #26266, #84022, #48027, #19169, #88443, #9357, #38241, #28162, #55631, #62756, #48983, #6849, #20587, #26745, #33847, #49457, #63695, #35723, #85437, #57053, #91588, #78345, #64637, #84480, #77881, #93465, #21501, #92520, #56584, #19630, #35246, #85889, #93004, #63224, #71722, #5449, #70777, #48499, #41386, #20101, #64172, #77398, #70319, #28618, #21041, #57507, #34318, #92056, #13028, #86351, #27686, #27210, #50379, #79283, #14424, #12535, #41864, #69827, #4962, #56097, #84951, #5910, #34780, #13487, #49909, #42334, #71245, #78804, #13949, #6374, #42806, #30006, #22427, #86821, #88672, #23821, #9127, #65094, #36635, #44191, #36175, #81565, #30461, #58891, #73096, #59356, #52232, #194, #79735, #87737, #51299, #21979, #52684, #65556, #57967, #44662, #29075, #72631, #670, #73563, #8226, #7751, #38004, #66914, #8672, #37104, #59831, #43731, #29554, #51759, #50852, #66013, #58434, #37550, #80648, #14877, #15331, #23365, #15803, #87280, #66461, #80192, #43281, #1125, #1579, #22889, #16258, #88208, #81115, #2052, #45108, #72179, #7295, #74010, #30943, #18118, #74472, #17193, #17661, #25676, #26143, #82512, #54093, #32331, #10996, #90977, #76353, #46514, #62148, #61681, #46054, #33251, #11479, #68786, #2524, #9603, #89589, #47444, #61233, #67396, #38491, #90068, #10531, #40329, #25220, #3916, #31401, #82965, #69245, #60291, #24760, #4373, #55038, #39398, #3436, #89128, #75872, #32792, #39865, #10072, #18578, #74960, #75415, #24279, #82035, #60749, #90512, #53154, #38940, #16713, #54555, #45568, #67849, #2975, #53643, #31860, #68313, #46970, #83423, #13830, #28499, #62634, #34202, #34663, #27562, #40792, #71124, #20923, #26624, #48855, #48380, #35122, #85319, #19059, #91474, #11943, #56457, #71599, #83907, #63107, #55515, #92402, #27089, #55976, #76817, #49792, #20469, #64523, #12909, #78230, #47914, #77760, #64043, #19979, #41747, #78689, #5334, #49336, #13369, #70660, #4840, #91935, #42210, #69709, #92885, #6254, #5789, #84364, #33723, #19513, #84830, #63577, #28046, #77283, #56936, #12413, #85773, #42681, #93348, #6734, #35607, #41263, #70201, #58324, #57847, #73450, #9016, #86701, #37895, #51642, #59239, #43619, #50254, #72516, #15217, #21865, #36991, #88085, #23242, #37440, #50741, #8561, #66349, #87167, #1464, #52121, #1930, #44073, #72975, #57391, #79625, #58779, #65436, #80528, #15681, #7187, #86233, #44547, #16146, #81003, #44998, #14766, #14308, #21385, #1016, #72070, #7636, #36520, #73900, #79161, #550, #43169, #30350, #22773, #36062, #8104, #66800, #22316, #64979, #82, #51187, #29433, #28961, #80074, #65903, #29895, #87622, #17549, #89016, #9959, #89957, #24163, #52575, #61574, #82401, #16604, #53044, #31292, #75764, #59721, #81919, #81455, #39284, #10420, #88564, #89478, #53986, #67738, #30824, #23712, #24638, #45938, #2412, #45459, #38831, #53525, #46401, #61118, #2864, #75301, #39747, #68202, #32212, #60178, #18007, #32688, #17071, #3322, #74846, #10884, #25112, #9482, #31748, #67282, #82855, #74359, #38368, #46860, #68672, #60640, #3807, #87460, #14605, #81299, #59078, #2250, #44384, #15991, #50576, #80370, #66644, #51482, #73294, #16445, #36829, #51951, #87921, #15511, #36362, #857, #23072, #79471, #1770, #80842, #8406, #87008, #43463, #29268, #22607, #65748, #66190, #380, #29738, #79916, #44843, #8858, #31134, #45297, #1307, #74202, #22160, #37284, #51028, #37736, #67116, #15053, #60020, #73746, #23555, #7935, #72360, #58619, #30189, #43915, #30654, #52424, #9319, #59555, #72810, #88405, #38202, #21699, #7477, #65275, #58164, #46700, #10726, #88859, #53352, #90256, #3164, #18306, #47163, #38677, #24008, #76072, #47643, #54745, #76546, #81761, #33440, #11203, #39582, #24955, #40061, #4109, #16911, #31592, #75602, #68038, #67582, #40518, #17393, #9803, #25405, #74679, #24472, #46242, #54284, #53832, #82237, #83623, #18785, #83154, #82698, #11669, #89318, #75146, #3640, #2710, #89792, #10258, #68979, #32530, #45769, #60943, #32981, #61424, #39126, #61872, #60481, #69436, #32049, #90703, #68505, #25864, #17849, #4566, #52881, #34855, #91183, #71797, #13101, #69905, #63768, #26351, #62833, #63301, #71319, #6919, #34394, #5983, #77958, #56661, #42884, #28233, #92132, #14023, #13558, #91667, #78875, #57121, #78420, #48106, #55242, #41465, #93079, #41939, #19248, #84099, #70851, #56174, #85962, #92597, #42408, #77010, #27766, #21113, #12138, #70396, #49981, #62343, #85031, #49062, #40984, #85510, #6449, #35324, #55707, #64249, #84558, #27287, #5044, #33925, #12619, #19705, #48575, #77476, #5524, #20182, #12394, #82945, #54075, #68767, #41240, #76333, #90049, #48361, #77264, #63087, #3416, #3897, #5315, #84344, #46494, #18097, #25653, #76797, #68295, #24743, #11923, #70182, #19495, #34184, #75853, #75397, #53625, #62127, #39380, #32774, #46951, #82495, #17643, #39845, #10510, #47894, #83889, #61214, #69225, #91455, #83405, #25201, #10975, #54536, #61662, #90494, #18556, #47423, #11458, #40310, #90958, #4354, #33231, #33702, #26123, #55018, #19039, #40772, #55496, #69690, #4820, #62614, #26605, #93331, #27070, #5771, #19961, #64505, #79608, #36504, #71103, #34645, #6718, #35106, #64025, #84811, #57831, #35591, #72500, #20905, #86217, #55957, #56917, #43152, #28028, #49776, #86682, #13349, #28482, #57375, #85757, #12890, #6236, #21369, #48833, #72055, #50239, #78671, #63555, #77740, #92384, #92866, #42190, #42664, #70643, #13812, #56436, #79143, #14293, #7618, #21847, #71581, #50723, #27544, #7171, #85300, #36046, #43604, #20448, #91916, #64963, #64, #78210, #41727, #28945, #14749, #49316, #44983, #2397, #31274, #45441, #58762, #16585, #74342, #1447, #9466, #60161, #9943, #23225, #80989, #65420, #29878, #66785, #73434, #88548, #23696, #52104, #38351, #51625, #15198, #24147, #37879, #532, #74831, #16131, #72958, #1915, #29417, #65888, #66334, #67265, #58307, #37423, #9001, #73883, #59705, #45921, #89000, #30332, #17056, #53025, #998, #81903, #87150, #52560, #51171, #22300, #44531, #80058, #30806, #44058, #8087, #81438, #59222, #36975, #87604, #22750, #80512, #15661, #8544, #88068, #46842, #69584, #84242, #32673, #25548, #2852, #4247, #26013, #62016, #32196, #40664, #68185, #39731, #60624, #10403, #82837, #33127, #31733, #39268, #4712, #54899, #26500, #3306, #61101, #17990, #55391, #90392, #89941, #62499, #91338, #77157, #17534, #75745, #19392, #33590, #89462, #25096, #68654, #24623, #38816, #83776, #54429, #3790, #18932, #47787, #53508, #75284, #83300, #10868, #82385, #48255, #53970, #46384, #40205, #61559, #18448, #47306, #69121, #76221, #11352, #67720, #90851, #76688, #11813, #30115, #12781, #41623, #20802, #91815, #13248, #70544, #71475, #49672, #34080, #78107, #86115, #78568, #5666, #13706, #48729, #58998, #20341, #92281, #63919, #34542, #85654, #44304, #73215, #21264, #63450, #57271, #50134, #42084, #79033, #8331, #51871, #92756, #27924, #12288, #27437, #42558, #49211, #35485, #64401, #55858, #41132, #93227, #66119, #37212, #1233, #56329, #62982, #70065, #6607, #26967, #85193, #71000, #87847, #5206, #6132, #84711, #28380, #15438, #19858, #56812, #22996, #35003 ),
 ( #77631, #53271, #68428, #25332, #59943, #88324, #89241, #23931, #52802, #73671, #46626, #24394, #61350, #9723, #75069, #15916, #45686, #31972, #16829, #38602, #75526, #2167, #17311, #82155, #74594, #1690, #88783, #46166, #44771, #60865, #10181, #67506, #52345, #8782, #23479, #81680, #31056, #31515, #59469, #2636, #45219, #39050, #67962, #90184, #10649, #60403, #39507, #81222, #3087, #16368, #89708, #32447, #74121, #80764, #24875, #82623, #67031, #37660, #9242, #53757, #17771, #66568, #3558, #30572, #38120, #48501, #34782, #20104, #84025, #5912, #5452, #83544, #70779, #48985, #12538, #39986, #47087, #33364, #84954, #4965, #11120, #18235, #33849, #48029, #77884, #69829, #41388, #75991, #62758, #13031, #68903, #62265, #41866, #63697, #76934, #40909, #4035, #19632, #70321, #77401, #47566, #56099, #18702, #55162, #32907, #25789, #4487, #34320, #61795, #54671, #92523, #63226, #54211, #76472, #11592, #91099, #83080, #12062, #40440, #90627, #69357, #26268, #19171, #91592, #26747, #55633, #84483, #92058, #27212, #20589, #66016, #14880, #43285, #57509, #43734, #36639, #49459, #64174, #14427, #6851, #71248, #73100, #49911, #42336, #29080, #13489, #57055, #78806, #57971, #86354, #85891, #87283, #22430, #86824, #21505, #44195, #28165, #21043, #36178, #6377, #28620, #13952, #21982, #65097, #78347, #93467, #7754, #197, #42809, #50856, #93006, #8229, #35726, #79738, #72182, #673, #71724, #35249, #80195, #72634, #56586, #37107, #7298, #64639, #65560, #85439, #29557, #50383, #79286, #27689, #58438, #51302, #15334, #80652, #30464, #52235, #2527, #30946, #59360, #60752, #89593, #60294, #88675, #17664, #1582, #88212, #9607, #15806, #2056, #23368, #89131, #38494, #22892, #66918, #74963, #67399, #81118, #31404, #37553, #46517, #9130, #24282, #81568, #67852, #16261, #44665, #53646, #53157, #30009, #10534, #45571, #8675, #82039, #58894, #45111, #59834, #10075, #39401, #23824, #17196, #16716, #46057, #75418, #24764, #52687, #1128, #38943, #74013, #87740, #82516, #2978, #73566, #51762, #38007, #31863, #74476, #66464, #32335, #19062, #62151, #5337, #83910, #26628, #90071, #47917, #34205, #61236, #76356, #63110, #19982, #90980, #55042, #25223, #33727, #55518, #91477, #61684, #70205, #3919, #69248, #54096, #39869, #18582, #62638, #82968, #68789, #91938, #84367, #55979, #32795, #90515, #47448, #84833, #26147, #25679, #27092, #48859, #12912, #46973, #11482, #77764, #68316, #18121, #54558, #4376, #75875, #3440, #19516, #76820, #33254, #48383, #77286, #11000, #83426, #40332, #11946, #40795, #69712, #4843, #12416, #41267, #7190, #50257, #63580, #13833, #21869, #79165, #42213, #14312, #78233, #58327, #49795, #64982, #28502, #14769, #28049, #85323, #554, #43172, #70663, #51190, #86236, #49339, #72073, #5792, #71127, #42684, #50744, #80077, #71603, #36065, #57394, #85, #22319, #7639, #6738, #87170, #86704, #6257, #41750, #36523, #28965, #27565, #34666, #20926, #72519, #21388, #92405, #56461, #57850, #35610, #65439, #79628, #43622, #20472, #29437, #13372, #35125, #78692, #64047, #92889, #64526, #56939, #85776, #93351, #2415, #38372, #8564, #17074, #44550, #16149, #36995, #80531, #59242, #74362, #72978, #15685, #74850, #31295, #2867, #73453, #37443, #88088, #31751, #66803, #66352, #38834, #67741, #53529, #87625, #23246, #89481, #9962, #65906, #1467, #45001, #8108, #15220, #60181, #30828, #73903, #89019, #24166, #1020, #51645, #1933, #52125, #58782, #60643, #30353, #29898, #16607, #22776, #81006, #9019, #45462, #37898, #59725, #24641, #44076, #9485, #88567, #67286, #23715, #52578, #81922, #81458, #53047, #45942, #83319, #46863, #3325, #17552, #39750, #18465, #54446, #54915, #68676, #47324, #91357, #33144, #26032, #39287, #69600, #19409, #25115, #76240, #75767, #33608, #83795, #46404, #89961, #10423, #18950, #70081, #26984, #61577, #53989, #90868, #25566, #11372, #75304, #48272, #47804, #62999, #40222, #76705, #68206, #69138, #62516, #4266, #62034, #77174, #3811, #11831, #40682, #4730, #32215, #90409, #26518, #61122, #55406, #84259, #12304, #82858, #18010, #10887, #41148, #32691, #5224, #34097, #91829, #82405, #86130, #43062, #65335, #50635, #35501, #79525, #27452, #56830, #56344, #71967, #7533, #85206, #36418, #50152, #57745, #42100, #48744, #71015, #13722, #20357, #64417, #86589, #21760, #35957, #49229, #7085, #64876, #85670, #93702, #14664, #439, #42575, #71490, #55873, #78125, #57288, #63933, #79050, #14201, #5683, #84725, #28858, #43519, #72417, #19874, #13263, #12799, #77648, #93243, #70559, #6147, #35019, #41641, #34557, #92771, #63466, #92295, #27939, #20818, #49688, #78583, #6621, #28396, #21279, #59132, #1359, #1825, #80425, #87976, #38258, #73799, #66697, #79970, #16499, #60074, #65800, #23127, #87516, #74253, #30711, #58219, #36885, #51082, #59610, #16963, #67634, #8458, #912, #37790, #66244, #30242, #22212, #88911, #88460, #9854, #52010, #23608, #87064, #80897, #9376, #16044, #44896, #24061, #44440, #52475, #81349, #8913, #43967, #37338, #45351, #15107, #67172, #2305, #31189, #29791, #72867, #58671, #52937, #73346, #81814, #7992, #45827, #22662, #74733, #38728, #29326, #51535, #15569, #91242, #68091, #3699, #3217, #18842, #48157, #32106, #77061, #90760, #4619, #82748, #89370, #17901, #54339, #61004, #76128, #33493, #62401, #76599, #89849, #47699, #11720, #32584, #40574, #26407, #41033, #83212, #18359, #2761, #25011, #4162, #10778, #25918, #54803, #46293, #31642, #83680, #55296, #84150, #19298, #53882, #53407, #60532, #40115, #17443, #46754, #75655, #12190, #24527, #39640, #82292, #69488, #61924, #75197, #47219, #10310, #61476, #11262, #68564, #39180, #90306, #25459, #69030, #33033, #50510, #35840, #91718, #63353, #70900, #62884, #14544, #57172, #85557, #6034, #86012, #78926, #26871, #12680, #56711, #49114, #19760, #21632, #92184, #84611, #71370, #55758, #5574, #27339, #6502, #34906, #34445, #64757, #93582, #35381, #63817, #86467, #70447, #56226, #78470, #48628, #92651, #85088, #64301, #13607, #77530, #41987, #50031, #42460, #20237, #93126, #41521, #79408, #78011, #28281, #20705, #42938, #13151, #27821, #28741, #21162, #5101, #69961, #49575, #14075, #71847, #33981, #6967, #57624, #52359, #52815, #15450, #80780, #59013, #37674, #23943, #9255, #73232, #88795, #88340, #72749, #59957, #38132, #1703, #29201, #36296, #22547, #74137, #87860, #317, #7414, #23009, #37227, #67047, #51888, #30586, #65213, #15930, #2183, #58099, #51421, #31069, #81695, #66132, #30129, #86947, #8795, #59488, #66583, #36760, #45232, #7870, #44321, #22099, #14992, #87400, #23492, #50969, #43851, #43399, #81235, #72294, #65680, #795, #80311, #79853, #16382, #29675, #8344, #58556, #1247, #44784, #73685, #31983, #47099, #83092, #10662, #31527, #89724, #18247, #45699, #91958, #54224, #39518, #82170, #9739, #24406, #17784, #60876, #61361, #89255, #24887, #75082, #76006, #5357, #27585, #12931, #90195, #41771, #17326, #46637, #46177, #34223, #63599, #10192, #92423, #11137, #20002, #3100, #38615, #53768, #68439, #39061, #25343, #48880, #77783, #27113, #67973, #63129, #55997, #75538, #84852, #70681, #56482, #3572, #32461, #16843, #82634, #41287, #70222, #5811, #34685, #60415, #74611, #67519, #2649, #53285, #65455, #20943, #13389, #87186, #14328, #71145, #13850, #85792, #7655, #20491, #78708, #42232, #102 ),
 ( #49811, #57867, #72089, #49357, #35143, #78251, #7206, #572, #85340, #57413, #42703, #28981, #86252, #21403, #92906, #58344, #86723, #6274, #36081, #21887, #64066, #56955, #43188, #28066, #71621, #43638, #36540, #64542, #6754, #35627, #93368, #50759, #28518, #79643, #29456, #65000, #14785, #72536, #50276, #79184, #76667, #42064, #63430, #63896, #40644, #11794, #26479, #92732, #34057, #47768, #6111, #34982, #20781, #54878, #55369, #56792, #70978, #4230, #69564, #77136, #69104, #76204, #92259, #91793, #12267, #27416, #85170, #33108, #18913, #62959, #84221, #25992, #27904, #4692, #90832, #77608, #61997, #33567, #62477, #12759, #41109, #91318, #85634, #11333, #41600, #70041, #40185, #19368, #48233, #84687, #83757, #5183, #26944, #70522, #19836, #55832, #48704, #56304, #5648, #34523, #20321, #49191, #78086, #13229, #72827, #36380, #22623, #35920, #93207, #8421, #22176, #78547, #59095, #397, #57251, #51044, #13685, #50112, #50595, #58634, #87936, #21720, #87025, #65293, #43930, #30204, #15527, #79489, #1322, #874, #79007, #66206, #44402, #7952, #35463, #42537, #28823, #80385, #29287, #6585, #71448, #58183, #43482, #73310, #79932, #36847, #64382, #15068, #28359, #86093, #21243, #65764, #37300, #49653, #57706, #14162, #29753, #86549, #14624, #43026, #71929, #87475, #7051, #72378, #51497, #64838, #7495, #93663, #52896, #74696, #17864, #38218, #53367, #89332, #16925, #37751, #2267, #24487, #51969, #3180, #60495, #45784, #88422, #16006, #30669, #24022, #67133, #67598, #1786, #31150, #81313, #82253, #10273, #32548, #46716, #2726, #75618, #23571, #81775, #52438, #39142, #68522, #16459, #3659, #17408, #24973, #9335, #44858, #60036, #9818, #45311, #31606, #53847, #82713, #32064, #74216, #68053, #60959, #38691, #89811, #10742, #61441, #46256, #75160, #23087, #88873, #39599, #80859, #73761, #8873, #66659, #59572, #77492, #49078, #56191, #77977, #47661, #47179, #34871, #33944, #11223, #40536, #83639, #20199, #54300, #11685, #76089, #19722, #55722, #83173, #40998, #63317, #55258, #90271, #25422, #91200, #54762, #40078, #18323, #76562, #26369, #62359, #62849, #69451, #84113, #5539, #69921, #91683, #68995, #12637, #27303, #32997, #19263, #18803, #41484, #26834, #4126, #61888, #90720, #84574, #13118, #25881, #4581, #33456, #5061, #48121, #77025, #12153, #85050, #48592, #70867, #70414, #34410, #92148, #41954, #5998, #93549, #21595, #58527, #78892, #288, #36265, #57592, #78438, #42901, #65185, #92614, #43820, #7384, #86436, #35343, #56678, #71336, #64722, #14039, #14515, #42424, #71815, #28250, #29169, #50941, #73196, #87372, #43370, #22520, #64267, #28707, #93096, #79823, #15421, #57138, #44289, #58064, #65649, #49997, #85526, #6935, #50475, #85979, #72266, #763, #29648, #72719, #21129, #14964, #7842, #79378, #36729, #51391, #8316, #86918, #22071, #63784, #35808, #80282, #27784, #20672, #49543, #13574, #6466, #24380, #89694, #3074, #24861, #88307, #87831, #75512, #74580, #51856, #81209, #30558, #60852, #1217, #52331, #22982, #60390, #2623, #30101, #81668, #10168, #2152, #37198, #66106, #38107, #1676, #80748, #58983, #23465, #67017, #9227, #9708, #16354, #31042, #46153, #16815, #38589, #15900, #53258, #67950, #73657, #59932, #59456, #82141, #88771, #31958, #52789, #89228, #44757, #45674, #53744, #8768, #45205, #82610, #17757, #23918, #67492, #37646, #31501, #17297, #75057, #74107, #39037, #66555, #46610, #32433, #75977, #54655, #69812, #68415, #11105, #70306, #91575, #92041, #68886, #39971, #83529, #27195, #62247, #4017, #34304, #63210, #48968, #83066, #18688, #84935, #5437, #61333, #32892, #11576, #3545, #10634, #26731, #26253, #40425, #55618, #19617, #90170, #47070, #91082, #47551, #54197, #56083, #61779, #25318, #12047, #18220, #90612, #25773, #40894, #69342, #76456, #20087, #39493, #4948, #4473, #33350, #55147, #84009, #19157, #48013, #76918, #33834, #62743, #84466, #48485, #77384, #12522, #41372, #78331, #50365, #20571, #655, #85874, #7281, #64622, #50838, #64156, #27672, #36618, #79268, #13014, #87265, #28602, #85423, #14409, #41850, #13472, #13932, #86807, #22410, #49894, #21485, #93448, #72165, #58418, #43716, #42790, #29539, #29060, #71231, #77864, #72615, #36158, #63680, #70763, #57036, #14863, #57492, #34766, #5895, #86335, #49443, #43267, #21025, #71707, #92504, #7737, #65080, #56570, #6834, #179, #6357, #35708, #57952, #21964, #79721, #65540, #92989, #35231, #28147, #45091, #65997, #30444, #23804, #80175, #31383, #88655, #73992, #22871, #44172, #58873, #52215, #66442, #2034, #29990, #1561, #15785, #81547, #38472, #60732, #46037, #30924, #74942, #51736, #81098, #80629, #67376, #2957, #44644, #31842, #45551, #53135, #37531, #73079, #59336, #9110, #73545, #59814, #82016, #17173, #60273, #8654, #2505, #89109, #16241, #24261, #10052, #89571, #37986, #66894, #51282, #88188, #52667, #23347, #74451, #9584, #1108, #15313, #38922, #67831, #8210, #37088, #16695, #87720, #22643, #20451, #91457, #27073, #70184, #7972, #40775, #91918, #33705, #7513, #42193, #69693, #27546, #51062, #41731, #76800, #11926, #77742, #41242, #26608, #4822, #34186, #12893, #48836, #49318, #63090, #70645, #87044, #56438, #78213, #62617, #65312, #15087, #19497, #5773, #5318, #29306, #13352, #55499, #84348, #48363, #71105, #65781, #77267, #55959, #36398, #12396, #84813, #43947, #419, #890, #19963, #34647, #63558, #29773, #92386, #85302, #36866, #58652, #58200, #22193, #79949, #87494, #72844, #73328, #44877, #52457, #44422, #89833, #38710, #67153, #81331, #67617, #60516, #8439, #87955, #38239, #30691, #1340, #3200, #73779, #66226, #52917, #37318, #80879, #8894, #81796, #16478, #16026, #17427, #46276, #16944, #45334, #68075, #51991, #37772, #60055, #30223, #74235, #66678, #45808, #88893, #59114, #23590, #31625, #24042, #1805, #74717, #23108, #32084, #59591, #9837, #2286, #24508, #88441, #9355, #10293, #2745, #80403, #60985, #31169, #89352, #53390, #15550, #82275, #75180, #39163, #51515, #90743, #62379, #40557, #19283, #5560, #84594, #54783, #70434, #69941, #54320, #41506, #19744, #77044, #10762, #17884, #4146, #55742, #69471, #75639, #82732, #4603, #18826, #48612, #33476, #12175, #46736, #91224, #77512, #39620, #33017, #12661, #34431, #47681, #11705, #68544, #84133, #41018, #48142, #18343, #26854, #83195, #25901, #3683, #90291, #69015, #63337, #83662, #26391, #55279, #5084, #24994, #53866, #76582, #32568, #33965, #47198, #61460, #25443, #62869, #76112, #11245, #61908, #40099, #91702, #49100, #56211, #42922, #85999, #29185, #14058, #50494, #20222, #71836, #58082, #85070, #6486, #86935, #43836, #21148, #78911, #77998, #57610, #79395, #21611, #85544, #305, #27805, #93114, #13138, #63804, #42445, #86453, #41974, #92633, #22087, #14531, #79840, #56698, #20692, #71355, #14980, #50018, #49562, #50957, #72738, #36745, #70888, #35365, #7858, #92168, #6018, #78457, #28269, #34893, #27325, #43386, #6954, #57158, #72281, #7401, #13593, #64286, #35827, #64741, #93568, #28725, #36282, #65202, #67032, #51408, #1235, #22998, #2168, #1692, #30117, #31517, #60405, #31057, #59471, #82157, #66121, #59000, #74122, #80300, #66570, #87849, #59944, #9243, #87389, #37662, #45688, #38121, #51873, #88784, #8333, #17313, #73673, #23932, #52347, #38604, #80766, #15440, #24396, #52804, #781, #75070, #16369, #73217 ),
 ( #16831, #81682, #29664, #37214, #22536, #74596, #53273, #10182, #44773, #15918, #9725, #8784, #30574, #58544, #89243, #67508, #46167, #88326, #2638, #44306, #23480, #65667, #81223, #45220, #33850, #54212, #69358, #11593, #32908, #53758, #18236, #40441, #67963, #19172, #76473, #61796, #10650, #31973, #46627, #39987, #83081, #83545, #17772, #47088, #3559, #4488, #26269, #48502, #62759, #18703, #91593, #39508, #68904, #68429, #55163, #84484, #32448, #19633, #33365, #40910, #25333, #60866, #75992, #90628, #61351, #47567, #69830, #4966, #48030, #90185, #84027, #76935, #4036, #12063, #26748, #77402, #25790, #54672, #39051, #11121, #62266, #91100, #55634, #3088, #82624, #89709, #24876, #75527, #72183, #198, #63698, #63227, #50857, #49912, #27213, #56587, #5913, #36179, #70322, #27690, #92059, #35727, #71725, #5453, #57056, #79287, #71249, #12539, #34321, #85892, #14428, #6378, #41389, #56100, #13490, #70780, #84955, #20105, #92524, #42337, #78348, #78807, #85440, #35250, #21506, #21044, #13953, #48986, #93468, #43286, #77885, #64175, #34783, #57510, #42810, #13032, #41867, #20590, #6852, #29081, #49460, #93007, #28166, #64640, #28621, #86355, #50384, #7299, #65098, #86825, #57972, #21983, #14881, #44666, #30947, #15808, #37554, #74477, #1129, #16262, #52237, #73567, #674, #58895, #81119, #43735, #59835, #23369, #8676, #51303, #72635, #87284, #80653, #30010, #30465, #58439, #87741, #44196, #45112, #66919, #89132, #9608, #59361, #38495, #80196, #66465, #15335, #2057, #31406, #73102, #60295, #74014, #81569, #66017, #7755, #22893, #1583, #8230, #88213, #16717, #45572, #88677, #37108, #23825, #52688, #9131, #67400, #2528, #24283, #38008, #79739, #36640, #51763, #65561, #29558, #22431, #11483, #2979, #53158, #40333, #11947, #19063, #40796, #10536, #10076, #91478, #90516, #67854, #3441, #46518, #76821, #17197, #68317, #38944, #76357, #18583, #25224, #25680, #68790, #47449, #33728, #47918, #82969, #4844, #4377, #82517, #69713, #62640, #69249, #31864, #46058, #32336, #83911, #3920, #60753, #74964, #32796, #46975, #82040, #61685, #33255, #89594, #54559, #24765, #53647, #61237, #17665, #75419, #75876, #39870, #39402, #62152, #90981, #26149, #90072, #55043, #54097, #18122, #11001, #83428, #70664, #85777, #84368, #27093, #86237, #13834, #14313, #84834, #55980, #5793, #43173, #78234, #91939, #50258, #79166, #64983, #5339, #34667, #7191, #21389, #48384, #19983, #27566, #19517, #26629, #42685, #42214, #56463, #71604, #35612, #77287, #63111, #13373, #63581, #70206, #72075, #48860, #41268, #28050, #12417, #77765, #12913, #56940, #85324, #41752, #36066, #55519, #20927, #20473, #34206, #92406, #49340, #35126, #71128, #6258, #64048, #49796, #92891, #78693, #6739, #64527, #93352, #28503, #57395, #36524, #16608, #8109, #23247, #80532, #66804, #80078, #43623, #52579, #66353, #28966, #9486, #44551, #7640, #1468, #57851, #555, #1021, #9020, #38373, #52126, #21870, #73454, #30829, #86705, #36996, #59726, #45463, #87627, #15686, #50745, #59243, #81007, #16150, #87171, #1934, #29438, #29899, #79629, #65440, #44077, #88089, #14770, #58328, #88568, #45002, #81459, #22320, #51191, #72979, #74363, #51646, #15221, #23716, #86, #72520, #65907, #58783, #22777, #8565, #37444, #30354, #73904, #37899, #11832, #54447, #82859, #3326, #83320, #76241, #60182, #9963, #53990, #46405, #17075, #18951, #89482, #81923, #68677, #53048, #2868, #24642, #3812, #32216, #31752, #33145, #62035, #32692, #61123, #83796, #67742, #60644, #75768, #45943, #68207, #53530, #61578, #10888, #89020, #39288, #47325, #39751, #82406, #90410, #38835, #47805, #75305, #25567, #18011, #40223, #17553, #74851, #26033, #18466, #2416, #76706, #46864, #10424, #11373, #31296, #89962, #25116, #69139, #67287, #4267, #90869, #54916, #24167, #21280, #6622, #70560, #86131, #85671, #70082, #57289, #35502, #92772, #26519, #33609, #19875, #71491, #85207, #91358, #4731, #20358, #34558, #64418, #56345, #69601, #5684, #20819, #63467, #92296, #93244, #55874, #71016, #13264, #27453, #55407, #48745, #42101, #62517, #49689, #78126, #49230, #12305, #84260, #48273, #41642, #84726, #6148, #19410, #77649, #5225, #35020, #27940, #50153, #28397, #63934, #79051, #41149, #56831, #34098, #78584, #40683, #63000, #77175, #13723, #42576, #26985, #91830, #12800, #65801, #43520, #87517, #44897, #73800, #87977, #7534, #59133, #23129, #43968, #52011, #8914, #52476, #913, #29792, #14202, #72418, #15571, #22213, #37339, #66245, #57746, #43063, #1360, #66698, #37791, #1826, #65336, #64877, #71968, #51536, #28859, #58220, #36419, #30713, #7086, #29327, #93703, #30243, #73347, #35958, #58672, #80898, #72868, #86591, #21761, #15108, #441, #50636, #79526, #87065, #7993, #79971, #80426, #51083, #36886, #16045, #22663, #44441, #14665, #59611, #88461, #8459, #23609, #45830, #33862, #84038, #16500, #88912, #9378, #55178, #70337, #27226, #60533, #24062, #91113, #24528, #53409, #74254, #48513, #26282, #63241, #10311, #76948, #3218, #40923, #38260, #62278, #19645, #45352, #89371, #77414, #34335, #75198, #68092, #67173, #48043, #69843, #12075, #74734, #84499, #16964, #82293, #2306, #52938, #31643, #4977, #31190, #81815, #12552, #62773, #5464, #9855, #38729, #17444, #92072, #39181, #67635, #41402, #81350, #60075, #2762, #46294, #32107, #19183, #91605, #26761, #55646, #49000, #691, #43301, #71740, #85906, #72198, #65113, #77899, #92536, #42825, #35262, #5926, #7772, #78362, #70791, #57525, #41880, #85454, #13502, #86370, #21058, #20602, #22001, #50872, #21521, #49925, #72650, #56600, #49472, #64654, #34796, #57068, #42350, #50399, #93483, #13043, #28178, #36194, #28636, #71263, #79304, #27702, #36656, #64188, #14445, #6867, #29096, #6391, #63711, #14895, #7315, #84966, #65577, #35741, #93021, #216, #20117, #78822, #13967, #57989, #56114, #86842, #79754, #43750, #23843, #10095, #89154, #59379, #74983, #74496, #58911, #46077, #24303, #81590, #15351, #22446, #8694, #60316, #74033, #80211, #87300, #9150, #23387, #53180, #2075, #66034, #38963, #37574, #52709, #16281, #2548, #15826, #73118, #82059, #30966, #58456, #67875, #38028, #37126, #59854, #51319, #30028, #30484, #38514, #29575, #1601, #66937, #45132, #16738, #44211, #17216, #88231, #8245, #9628, #87757, #1147, #22910, #45594, #51781, #80670, #66485, #44683, #88695, #73585, #52256, #67419, #81137, #31427, #18605, #55063, #24785, #76377, #33749, #60774, #11021, #62661, #48404, #90536, #83450, #89614, #62172, #83932, #26172, #90092, #4866, #32357, #3942, #53667, #68339, #46995, #91003, #82536, #3462, #91495, #19084, #84389, #61257, #25244, #75897, #19538, #54579, #54118, #26650, #55540, #41290, #75439, #39891, #77307, #12439, #17685, #82991, #32815, #46537, #2998, #47938, #47470, #61705, #76841, #11968, #10557, #39422, #11503, #68812, #18141, #31884, #25697, #40352, #4398, #69269, #33275, #40816, #69733, #49360, #41774, #28522, #57417, #85795, #13392, #79188, #77786, #12934, #92909, #27116, #20493, #70684, #20946, #28069, #63132, #78254, #71624, #56958, #5814, #34688, #50280, #86256, #78711, #56000, #34226, #27588, #93372, #35146, #91961, #5360, #64069, #42235, #21407, #6277, #13853, #84855, #49814, #14332, #20005, #56485, #43192, #72092, #71148, #42706, #48883, #6757, #35630, #64546, #63602, #70225, #92426, #85343, #82821 ),
 ( #5650, #48236, #76669, #90834, #77138, #70043, #53954, #3771, #47770, #40187, #10850, #12761, #83285, #75728, #62479, #46826, #90377, #18430, #91320, #25994, #25533, #26946, #55835, #26481, #54880, #77610, #61544, #54413, #69566, #39715, #61999, #47288, #55371, #4694, #17974, #33111, #41111, #33569, #76206, #84223, #32656, #41602, #69106, #19370, #11796, #34059, #11335, #68639, #19838, #12269, #89924, #70524, #40647, #4232, #5185, #25080, #83759, #18915, #62961, #61082, #91795, #84690, #48706, #28825, #15071, #399, #64384, #79934, #79491, #35465, #56306, #6113, #78550, #93666, #92261, #34984, #29289, #21722, #22178, #92734, #63898, #13687, #51046, #86096, #27906, #58185, #87027, #72829, #13231, #42539, #43932, #34525, #85172, #56794, #93209, #27418, #63433, #50598, #50114, #28361, #14626, #43484, #20323, #70981, #21245, #71450, #78088, #49193, #85636, #42066, #35922, #20783, #49655, #6587, #64840, #57253, #79009, #14164, #43028, #57708, #71931, #7053, #86551, #72380, #7497, #36382, #65295, #37302, #67135, #16461, #29755, #73763, #81777, #45314, #8423, #74218, #44404, #24489, #16008, #31152, #88424, #74698, #87938, #51499, #60498, #9337, #36849, #17410, #52440, #15529, #38220, #65766, #66208, #8875, #16927, #46258, #37754, #2269, #23573, #60038, #82255, #67600, #66661, #53369, #52899, #1324, #7954, #2728, #88875, #87477, #876, #80861, #38693, #81315, #58636, #22626, #24024, #1788, #31608, #45786, #9820, #80387, #89334, #73312, #30207, #44860, #59097, #23089, #30671, #51971, #59574, #40538, #62361, #4584, #68524, #77027, #10744, #33458, #3182, #54764, #12156, #39145, #83176, #41000, #26836, #68997, #61890, #68056, #69453, #91202, #26371, #3661, #69923, #39602, #76091, #32066, #46718, #25424, #55260, #60961, #75621, #5063, #84115, #62851, #32550, #61443, #54302, #91685, #32999, #90273, #33946, #55724, #19725, #53849, #18325, #84576, #75162, #89813, #47181, #11225, #24975, #10275, #19265, #90723, #40080, #48123, #82715, #17866, #4128, #25883, #83641, #18805, #47663, #76564, #11687, #50000, #34412, #77979, #6000, #78894, #78440, #13120, #14517, #43372, #14041, #42427, #65187, #49080, #41956, #57140, #63319, #49545, #70869, #42903, #85981, #70416, #20674, #28709, #21131, #34874, #71817, #85052, #290, #56680, #6937, #35345, #21597, #63786, #92150, #7386, #35810, #77494, #58066, #28252, #56193, #64724, #12639, #92616, #13576, #57594, #86920, #71338, #93551, #64269, #86438, #29171, #36267, #6468, #48594, #50477, #27786, #41486, #5541, #79380, #27306, #20201, #1220, #52790, #66556, #72722, #79825, #1677, #15902, #81669, #37648, #22522, #88308, #58530, #38590, #30103, #45207, #8769, #88772, #8318, #65651, #74582, #23466, #50943, #31502, #30559, #29650, #52332, #14966, #51394, #22984, #31043, #60391, #87833, #59457, #81210, #16355, #2624, #16817, #51858, #67493, #67018, #80284, #22073, #45675, #74109, #7844, #43822, #58985, #9709, #9228, #36731, #765, #38108, #44759, #87374, #2153, #59933, #15424, #23919, #44291, #73198, #80750, #37200, #66108, #73659, #75978, #53260, #54656, #76457, #18689, #82611, #91083, #24862, #90171, #17298, #60853, #39494, #83530, #82142, #89696, #55148, #11578, #76919, #53745, #17758, #68416, #12048, #47071, #46611, #19158, #48015, #33835, #3075, #3546, #69813, #84010, #46154, #75513, #25319, #75058, #89229, #40426, #11106, #54198, #69343, #4474, #10169, #31959, #39973, #32435, #39038, #40895, #10635, #61334, #90613, #83067, #18221, #68888, #25774, #4018, #32893, #4949, #24381, #47552, #61780, #33351, #62248, #26254, #71232, #48486, #63682, #92042, #28148, #6359, #84468, #34767, #42792, #35232, #64157, #92505, #27197, #28603, #57493, #57037, #56571, #79270, #63211, #56084, #92990, #77385, #27673, #84936, #85875, #21026, #19618, #85424, #71708, #49895, #20088, #78790, #5438, #14410, #70764, #13933, #49444, #35709, #48969, #12523, #21486, #6835, #91576, #72166, #13473, #70307, #64623, #26732, #77865, #20572, #93449, #7282, #78332, #86336, #42321, #50366, #43268, #62744, #55619, #41373, #34305, #13015, #41851, #5896, #88190, #21967, #29062, #15315, #66896, #80631, #86809, #181, #15787, #29992, #2036, #51738, #23349, #57954, #44646, #30926, #50840, #44174, #59816, #81549, #58875, #22873, #79723, #1563, #52217, #59338, #29541, #37988, #65542, #37090, #14865, #7739, #80177, #30446, #43718, #36620, #88657, #81100, #23806, #657, #58421, #73081, #52669, #87722, #87267, #16698, #45553, #74453, #72617, #8212, #36159, #65081, #22413, #51284, #65999, #1111, #73547, #16243, #8656, #37534, #45093, #73995, #66444, #9112, #90051, #82498, #53138, #55021, #31845, #24263, #10978, #89111, #38925, #60734, #83891, #32314, #3900, #38474, #68298, #54539, #39383, #61217, #4357, #24746, #39848, #75856, #3419, #82018, #17646, #68771, #67378, #83407, #46954, #25204, #74945, #2507, #17176, #10513, #53628, #54077, #46040, #46497, #67834, #32777, #90497, #19042, #33233, #82947, #62130, #10055, #18100, #2959, #25656, #47898, #89574, #9586, #61665, #11462, #75400, #31385, #18559, #47426, #76336, #40313, #69228, #90961, #26125, #60275, #44360, #8382, #29243, #73270, #87896, #37713, #51005, #43890, #93168, #57663, #833, #7454, #22584, #51458, #42981, #28320, #80347, #51927, #59049, #80817, #50549, #50070, #57209, #36801, #14117, #43439, #86510, #23049, #86050, #14582, #78966, #15489, #58597, #21199, #72786, #66168, #58138, #71886, #7008, #356, #21673, #35880, #64797, #79446, #86984, #65250, #65722, #72335, #22137, #37262, #7911, #29715, #93621, #1284, #30166, #28779, #79892, #36336, #15966, #87438, #44820, #73723, #8835, #39099, #54258, #11175, #45742, #74176, #75121, #9778, #38653, #59530, #32500, #10231, #53326, #39555, #52857, #16421, #25378, #68011, #1742, #76046, #17366, #9293, #3140, #30629, #67091, #67557, #75577, #66619, #2686, #32021, #82211, #60919, #47134, #61397, #31566, #18279, #17820, #2224, #83128, #90229, #24927, #52398, #88379, #74653, #3613, #46217, #23529, #81275, #89765, #60457, #45273, #53804, #82672, #38176, #46674, #31108, #59995, #89292, #88834, #23984, #24446, #10698, #81735, #68477, #16884, #63273, #33414, #41911, #69407, #40956, #61847, #11642, #84069, #5495, #4083, #40489, #5956, #27260, #27739, #4538, #62314, #19219, #56635, #91640, #91154, #63741, #92568, #78392, #18758, #48077, #20632, #34830, #90678, #26320, #69877, #32954, #40036, #56147, #55680, #5016, #85001, #49036, #25838, #76519, #26794, #76982, #83595, #85485, #55215, #54718, #41438, #47616, #12111, #33898, #70370, #62805, #84531, #49502, #68952, #34368, #19678, #48547, #77448, #12592, #92106, #20155, #77932, #13075, #70824, #22030, #35296, #79338, #87328, #50899, #13998, #79783, #49958, #30057, #21550, #36685, #80241, #72228, #51811, #13533, #14473, #71773, #28209, #42381, #64683, #43331, #7342, #14925, #93509, #36223, #22477, #58021, #43779, #64223, #720, #44241, #78849, #65142, #6896, #58484, #72680, #71294, #21088, #93053, #7799, #1175, #6421, #86397, #42858, #65607, #50434, #243, #57097, #73151, #29606, #87790, #29125, #51350, #85937, #86876, #15378, #8275, #37155, #66063, #28666, #58940, #22939, #35770, #57552, #59886, #53211, #15855, #60806, #24334, #9663, #52287, #73614, #88265, #81623, #2109, #31456, #59411, #30999, #45163, #17250, #67905, #90124, #75467, #60345 ),
 ( #25275, #38547, #2578, #80704, #74063, #82091, #88726, #10126, #38992, #30514, #44713, #3029, #39451, #46569, #68368, #38061, #37602, #8725, #46110, #1633, #23874, #9182, #10589, #66513, #52741, #23422, #31914, #75014, #81167, #89183, #16311, #16771, #66970, #45625, #74530, #67450, #89646, #24816, #53700, #82567, #17715, #3497, #32389, #61289, #12349, #42624, #86179, #91875, #20407, #19919, #6676, #56879, #83021, #63044, #77221, #27988, #43111, #27, #34606, #27029, #63985, #92344, #27499, #48320, #21330, #92825, #36006, #78172, #49736, #18174, #49277, #35553, #85259, #13310, #50200, #70604, #85720, #20865, #42148, #70136, #63516, #78633, #41198, #64466, #13775, #71066, #55918, #5272, #84770, #56397, #5731, #6198, #34141, #35065, #48791, #71543, #93293, #64924, #79104, #28444, #14253, #77699, #57337, #12848, #72018, #7135, #41686, #54152, #23183, #30764, #15161, #21811, #44020, #80471, #58272, #8506, #59666, #88509, #8961, #22264, #73845, #37840, #58722, #66746, #23656, #67227, #15620, #44492, #28906, #87114, #30294, #36938, #52066, #80948, #72463, #57794, #16093, #81398, #52522, #16546, #80021, #79571, #86644, #66295, #43567, #72917, #51138, #45402, #50685, #8044, #14714, #44945, #88026, #7582, #73396, #1872, #87566, #36467, #29839, #65382, #494, #65852, #74301, #29378, #960, #9425, #38312, #22711, #51585, #37385, #1407, #59182, #53928, #67682, #25966, #54847, #40619, #74787, #46343, #76642, #61970, #24108, #89420, #3264, #88961, #2358, #83260, #17948, #32154, #18404, #11309, #52989, #38778, #82796, #75245, #45881, #47744, #24574, #17012, #3747, #81863, #31690, #53462, #32629, #61055, #60585, #90807, #83729, #61519, #89898, #18889, #2809, #82343, #10826, #9904, #25056, #17491, #90350, #39686, #10360, #68143, #76177, #68610, #39225, #25506, #46799, #11767, #75702, #54384, #47263, #69078, #40161, #4206, #31236, #33081, #60122, #78980, #20293, #77107, #70952, #33541, #70009, #70495, #78522, #14132, #41573, #13202, #85138, #63870, #50085, #35434, #5623, #21215, #20755, #5152, #86065, #64356, #27874, #55344, #62446, #48678, #6555, #49167, #26455, #91289, #78060, #63404, #93182, #42038, #56767, #84196, #6084, #28334, #19343, #77579, #57224, #69535, #92233, #56279, #48205, #34958, #85608, #92704, #62933, #71423, #34029, #41085, #34498, #91767, #49626, #4668, #26919, #12238, #13659, #55806, #84658, #19810, #12730, #27389, #42511, #22597, #73737, #8849, #23063, #36351, #87912, #51941, #72801, #80831, #37727, #81290, #848, #58610, #42997, #7468, #44373, #51019, #66181, #1298, #86523, #71903, #30180, #1758, #66633, #30645, #371, #93636, #7023, #80361, #57680, #86999, #65265, #59544, #35894, #58153, #28793, #59064, #8397, #64812, #87451, #15982, #7925, #21688, #50565, #43904, #29257, #79462, #14596, #22151, #36816, #15044, #15502, #79906, #65737, #44834, #51472, #73284, #43453, #88394, #23545, #72350, #29729, #37275, #52415, #17839, #45288, #23999, #38192, #82689, #4099, #54736, #89307, #52872, #24944, #53342, #82227, #9310, #76063, #53821, #90694, #39116, #10716, #74191, #75137, #61414, #46233, #68029, #11192, #31583, #46691, #75593, #10247, #31124, #24463, #39573, #67106, #90246, #68495, #3156, #81751, #2240, #16901, #17381, #60472, #60934, #88850, #32039, #74669, #3630, #32518, #25854, #40052, #89781, #68969, #45759, #32970, #61863, #16436, #9793, #25395, #60010, #38668, #67572, #2701, #54275, #83145, #18296, #47154, #5515, #19695, #70841, #92588, #76537, #26340, #70387, #62824, #33430, #35315, #12128, #4556, #85021, #69425, #19238, #40974, #20173, #48564, #48095, #49519, #78411, #49053, #77467, #6440, #84088, #76999, #92123, #62334, #84548, #69896, #77949, #27277, #11659, #55697, #63758, #56164, #5035, #13092, #55233, #64240, #91658, #41930, #34385, #56653, #33915, #91174, #42399, #5974, #18775, #93071, #63290, #26811, #34847, #47633, #12610, #41455, #27757, #28225, #85502, #20649, #13550, #71310, #83614, #40506, #86892, #8744, #8292, #86412, #73633, #22956, #15395, #42875, #49973, #36240, #87807, #7815, #14015, #21105, #36705, #50915, #51830, #72696, #44262, #78865, #65626, #80723, #71788, #65158, #15876, #37621, #79799, #43796, #6910, #22495, #73173, #80259, #50451, #58959, #21568, #58040, #35785, #28683, #7358, #51368, #64698, #57569, #44732, #37173, #66532, #79353, #14488, #261, #1651, #14941, #93524, #66081, #1193, #30074, #43346, #57113, #72243, #22046, #29144, #738, #29623, #85953, #58501, #87346, #90142, #17732, #18192, #88746, #59904, #74552, #47044, #82111, #2128, #54170, #83039, #68860, #9201, #9683, #11075, #25292, #52307, #23892, #31476, #23439, #30531, #46587, #46128, #60364, #75485, #39468, #81184, #66990, #17270, #38565, #74082, #75945, #52761, #45180, #31932, #16330, #81642, #16789, #60823, #89202, #45643, #39944, #59433, #89666, #24354, #88284, #31017, #67467, #39010, #38079, #53229, #2596, #24835, #67924, #75031, #10144, #10610, #3048, #53718, #82585, #68385, #3516, #32408, #61306, #84438, #70732, #83982, #47524, #56538, #70276, #32864, #13442, #48455, #11550, #5409, #61753, #4443, #4915, #12983, #42289, #69784, #41342, #19586, #92012, #78303, #63651, #33801, #49413, #48935, #33323, #20543, #92473, #56052, #83499, #90585, #76888, #34735, #77356, #54627, #25746, #12490, #91545, #27639, #34274, #84906, #18657, #63181, #85395, #76429, #12016, #3989, #40397, #26701, #27164, #69315, #62220, #62715, #91049, #77835, #20054, #26223, #55117, #19130, #41821, #47985, #40866, #55590, #5865, #79691, #14379, #43239, #64124, #37059, #14833, #51709, #149, #65503, #6328, #36129, #22380, #7253, #29029, #65969, #86305, #7705, #43687, #65046, #85844, #50330, #72583, #35196, #51253, #36589, #57916, #42756, #92960, #78761, #72137, #21457, #21934, #49862, #79237, #35680, #622, #58389, #80597, #1080, #50806, #29960, #71673, #86773, #6807, #87232, #22842, #64595, #15754, #29507, #73045, #57462, #28119, #80143, #15283, #93420, #44140, #8175, #58846, #87689, #28572, #71201, #57007, #20996, #13902, #39348, #82918, #2478, #60243, #44614, #9078, #46007, #52639, #67802, #2927, #88155, #73518, #31812, #3389, #10482, #32277, #2000, #1530, #8627, #81985, #59307, #88627, #37958, #68267, #37504, #59786, #30416, #60705, #10023, #66413, #89081, #17614, #9552, #23314, #52187, #45521, #66865, #81068, #16213, #30893, #74423, #16666, #17141, #23774, #38439, #53594, #24230, #74912, #45064, #89545, #73964, #67348, #81519, #31355, #53107, #38893, #24708, #82467, #61183, #46465, #90021, #75368, #25174, #54048, #34623, #69665, #83382, #41704, #70621, #56415, #90471, #62100, #92360, #77715, #39817, #11433, #19016, #10951, #18072, #5289, #33676, #47868, #34159, #27045, #68740, #54510, #4797, #90933, #61638, #63533, #40284, #32750, #19470, #3871, #47396, #69201, #48337, #76771, #76307, #12865, #5748, #77238, #11899, #27522, #18530, #4330, #26581, #25628, #40748, #33207, #12368, #55470, #26098, #83863, #91891, #84319, #54987, #41216, #62585, #46925, #91427, #70153, #63062, #84788, #55933, #19938, #75827, #48808, #20424, #2256, #36025, #92841, #86662, #49293, #85736, #86196, #513, #31139, #57355, #28923, #7150, #79589, #67121, #51153, #21348, #38207, #36483, #20882, #9324, #80037, #43583, #71083, #78188, #64484, #22281, #64942, #42168, #13326, #43, #79123, #15178, #57811 ),
 ( #43130, #49754, #21826, #44036, #72938, #65400, #78651, #29395, #58287, #50219, #87130, #85274, #6215, #72035, #50701, #35084, #13791, #14730, #93311, #72481, #7596, #64003, #28004, #56897, #42643, #71560, #6695, #35570, #28461, #14270, #3646, #74683, #10262, #53356, #83629, #24012, #75150, #16915, #83161, #25411, #52885, #10732, #32987, #24961, #4572, #60026, #60948, #24477, #9807, #88863, #17397, #89798, #32054, #32537, #46246, #53837, #68985, #39588, #61430, #45773, #47169, #90709, #2716, #82703, #82241, #11209, #90262, #81765, #67586, #38681, #54290, #47650, #31596, #39132, #60485, #68511, #3170, #17854, #89322, #25870, #18313, #40524, #46705, #76078, #68043, #75608, #40067, #4115, #61878, #54752, #18791, #76552, #11675, #69442, #48112, #12625, #5989, #62349, #13564, #70857, #56180, #5050, #26357, #40989, #34400, #48582, #77965, #12144, #77482, #91673, #63774, #20662, #42890, #28240, #13108, #57127, #33932, #63307, #62840, #56667, #20188, #6455, #19711, #77016, #85969, #34861, #91190, #71803, #41945, #69911, #92603, #55248, #26826, #92138, #42414, #33446, #5530, #27773, #49068, #85516, #14029, #93085, #27293, #78881, #78426, #55713, #49987, #21119, #49533, #19254, #84105, #41471, #64256, #71325, #84564, #70403, #35330, #85038, #58974, #36721, #15412, #93539, #754, #87823, #35799, #86907, #22973, #44747, #43811, #7833, #64712, #22512, #44280, #73188, #7374, #30091, #43361, #50931, #28698, #14504, #29159, #51383, #57583, #72257, #51845, #8307, #80740, #36255, #65174, #58056, #15891, #65640, #279, #73649, #8759, #6925, #22062, #14956, #86427, #21583, #79815, #72711, #29638, #58517, #50465, #79368, #87362, #80274, #37189, #66097, #1209, #34239, #78269, #70698, #41302, #43204, #20019, #12454, #92923, #77321, #27129, #48897, #28084, #27603, #56012, #57429, #86270, #56972, #85359, #14345, #91975, #84869, #6293, #70239, #92440, #77799, #85810, #35162, #19551, #63615, #71637, #64084, #12949, #20960, #63145, #72105, #5829, #6769, #84402, #41787, #13408, #34701, #5372, #7222, #56500, #20507, #49828, #49376, #42251, #71164, #78725, #13867, #42720, #21422, #50296, #35644, #64561, #36096, #93385, #28538, #79202, #91508, #26664, #55553, #48417, #73483, #86739, #37024, #45031, #8595, #65472, #37472, #7673, #81488, #73012, #88121, #51676, #37925, #51220, #14800, #23743, #66382, #116, #74390, #15719, #72551, #1498, #28997, #589, #65938, #73931, #9518, #1049, #30382, #80565, #59275, #45489, #30860, #29928, #16635, #16179, #29472, #65016, #59754, #23278, #50774, #57883, #44109, #1968, #44580, #21901, #79659, #52153, #58813, #88594, #81035, #9047, #43656, #66831, #52606, #36557, #8141, #58360, #87200, #87656, #22348, #80110, #15249, #22807, #61605, #31779, #40252, #67769, #39317, #60210, #9990, #82433, #3838, #2445, #38863, #4295, #25595, #26063, #2896, #60673, #17583, #54952, #89988, #89511, #62064, #90898, #76737, #17109, #46432, #18983, #33174, #89049, #24676, #68234, #31323, #38406, #54478, #54018, #3356, #83347, #18495, #53561, #47359, #76274, #32246, #11400, #83829, #67315, #25142, #82885, #24198, #75335, #39785, #10451, #90438, #69168, #81952, #53075, #47835, #74880, #61153, #18041, #46893, #75794, #10917, #68708, #32720, #55903, #5257, #64452, #69633, #27015, #62552, #35051, #71051, #4761, #56379, #78618, #70590, #11864, #40714, #12834, #70120, #26549, #33642, #63030, #41672, #77683, #78158, #91861, #5717, #20851, #85245, #49263, #91394, #92809, #42610, #48304, #34592, #34126, #56864, #13296, #55437, #19439, #84289, #42134, #93278, #77204, #84756, #12334, #20392, #48777, #63500, #41180, #71527, #6184, #86164, #92330, #63968, #19904, #27974, #85706, #49722, #13762, #6661, #28430, #57323, #21316, #72904, #12, #58257, #51572, #14239, #59168, #22697, #8028, #50671, #72002, #86627, #80006, #478, #29825, #57780, #29366, #43553, #15606, #66281, #88497, #73834, #58707, #8948, #79557, #15145, #14698, #1394, #30751, #72449, #59653, #73383, #80935, #65368, #7121, #87100, #36925, #7568, #87550, #16080, #44933, #36453, #22250, #1860, #65839, #51120, #37827, #66733, #23644, #21797, #44006, #79087, #43097, #35990, #947, #80458, #64910, #28891, #30278, #44478, #8493, #88014, #23169, #37371, #52052, #39214, #31678, #2346, #4196, #74774, #67213, #53917, #38298, #81850, #9891, #82785, #82330, #17000, #18395, #47252, #17937, #46331, #69067, #52975, #45868, #61042, #31224, #53449, #38766, #46788, #89885, #74288, #24562, #32619, #25045, #67670, #75690, #88949, #33071, #60572, #10815, #68129, #25496, #2796, #60109, #11298, #39677, #81386, #61961, #3253, #24096, #68599, #16534, #89408, #17480, #61509, #90797, #75234, #3735, #32143, #90341, #52510, #76166, #10348, #45387, #54374, #83249, #9412, #40151, #78049, #11757, #18878, #5140, #56752, #70483, #76633, #83718, #5611, #19799, #85595, #41560, #13190, #47734, #34486, #20742, #40609, #34018, #49613, #71411, #48668, #12719, #69525, #85127, #42025, #49153, #19333, #27861, #55334, #26908, #4656, #91278, #69999, #20279, #33530, #26443, #78508, #70940, #13646, #84185, #42497, #62436, #41074, #48195, #6071, #34944, #77097, #63392, #92691, #84648, #64341, #25956, #55796, #12227, #62921, #54837, #91756, #77569, #92222, #27377, #56267, #63858, #6543, #35421, #62317, #75579, #12113, #55682, #61399, #83597, #83130, #69880, #26322, #53806, #32502, #46676, #91157, #12594, #63275, #4085, #90231, #55217, #61849, #90680, #17823, #84533, #84071, #5497, #47618, #19221, #82674, #18760, #5019, #54721, #76521, #19680, #40038, #48079, #76984, #11644, #39557, #32956, #40958, #10700, #33900, #62807, #40491, #25380, #68479, #54260, #25840, #68954, #69409, #3615, #4540, #18281, #91642, #26796, #34370, #48549, #77450, #41440, #47137, #70372, #11178, #24929, #43781, #27741, #72682, #86399, #245, #78394, #85004, #13535, #49960, #56637, #71775, #29128, #58024, #72230, #85487, #43333, #7344, #28211, #36225, #86878, #36688, #78851, #14001, #92108, #20634, #93511, #6424, #21553, #50437, #41913, #27262, #79340, #50901, #22032, #79785, #49504, #49038, #56149, #35772, #13077, #42383, #71296, #35299, #6898, #77934, #93055, #64225, #57554, #64685, #20158, #57099, #65144, #28668, #92571, #14475, #34832, #14927, #85939, #7801, #42861, #70826, #21090, #5958, #63743, #38064, #722, #75015, #16313, #73154, #66973, #29608, #66066, #66516, #74534, #10128, #37604, #9186, #81169, #59888, #46112, #31459, #1636, #17253, #16773, #1178, #82093, #60348, #23876, #51352, #58486, #44716, #2580, #45165, #22479, #87331, #74066, #59414, #89185, #2112, #52744, #80243, #31002, #24338, #15380, #73616, #53213, #65610, #88268, #52290, #44244, #88728, #81625, #45627, #58943, #67452, #30059, #30517, #8277, #37157, #15857, #9666, #87792, #22941, #51814, #38549, #80707, #8728, #23424, #83023, #55576, #90570, #10591, #62700, #91530, #77342, #17716, #18176, #19572, #4900, #60807, #32392, #39928, #31915, #38994, #26207, #54612, #68846, #55101, #47971, #89648, #75469, #25729, #47027, #82568, #84424, #61291, #53701, #40383, #24818, #68370, #90126, #69301, #3974, #3500, #33786, #26687, #4429, #32849, #48440, #39453, #67906, #76414, #3031, #61738, #33308, #46571, #83483, #83968, #18641, #47508, #25277, #54154, #62205, #11536, #91035, #75930, #11058, #19116, #76875, #12002, #40851, #69770, #77820 ),
 ( #92461, #64108, #41808, #85831, #43226, #72126, #86291, #5851, #57450, #21445, #42275, #50318, #7242, #50795, #92946, #28106, #12476, #70719, #13889, #20530, #35667, #64582, #56037, #41326, #93407, #65035, #36118, #136, #63637, #63167, #70261, #49849, #27150, #56524, #34722, #29018, #5395, #27625, #91997, #28559, #71659, #34260, #56993, #79224, #71187, #84891, #20041, #13428, #85381, #48921, #12969, #49399, #6315, #78290, #78747, #35183, #20982, #14366, #42743, #6792, #57905, #86760, #21921, #22369, #44603, #44130, #30882, #81058, #14822, #87222, #7693, #52176, #67337, #24220, #58834, #51243, #88145, #22830, #51699, #72572, #43676, #59775, #23302, #8617, #80132, #36579, #15271, #80587, #1070, #30405, #58378, #29950, #73035, #16203, #66855, #89071, #74412, #59297, #9542, #8164, #15743, #37047, #1990, #31345, #65959, #60233, #73953, #81509, #87679, #65493, #73507, #37494, #66403, #45054, #16656, #45510, #88617, #1519, #23764, #52630, #9068, #38428, #2468, #79679, #37946, #612, #29495, #17604, #54500, #61173, #76297, #11422, #2917, #53095, #40274, #11887, #19004, #40737, #10472, #10013, #91416, #90461, #67792, #3379, #46455, #76760, #17130, #68256, #38883, #69190, #18520, #45996, #3859, #26087, #18062, #81974, #74901, #54038, #75357, #31801, #60694, #39338, #82908, #25164, #25618, #32267, #46915, #62088, #32739, #83370, #89534, #4320, #83852, #24698, #75816, #90009, #33197, #47384, #53582, #82456, #10940, #90921, #69654, #39807, #68729, #61628, #54976, #47857, #4784, #33664, #62574, #65267, #8399, #50568, #22153, #56769, #86525, #72803, #57682, #79464, #22599, #43001, #58156, #373, #21690, #42513, #7025, #29260, #57226, #78982, #87001, #14598, #86067, #87453, #51474, #51021, #43455, #44376, #28336, #21217, #36353, #13661, #28795, #50087, #79908, #15046, #49628, #93638, #7927, #43906, #14135, #36819, #64358, #73287, #35896, #65741, #72353, #850, #71905, #71425, #80363, #29731, #85611, #37277, #7470, #35438, #58612, #20757, #64814, #15504, #66183, #27877, #78524, #6558, #93184, #89309, #75595, #60936, #31127, #46693, #46235, #30647, #17841, #89783, #53344, #80834, #87914, #74193, #32041, #45762, #51943, #59067, #74671, #88852, #24947, #16903, #82229, #23065, #9796, #53823, #15984, #9312, #82691, #10718, #24001, #81753, #44836, #60474, #17384, #24465, #88398, #3158, #59547, #2243, #73739, #66635, #45290, #75139, #8851, #1760, #39575, #10250, #1300, #23547, #52417, #38194, #30182, #52874, #81292, #37729, #16438, #67108, #60012, #38670, #67575, #2703, #31585, #39119, #68031, #61416, #13094, #55699, #84090, #4558, #84550, #77469, #90248, #11194, #55235, #47635, #18298, #20175, #90696, #83147, #69898, #54277, #32522, #33917, #19697, #91660, #61865, #70389, #4101, #69427, #25397, #40055, #18777, #62826, #47156, #68971, #34387, #48566, #56166, #32972, #25856, #76539, #85023, #26342, #54738, #92125, #27279, #68497, #76065, #11661, #49055, #63292, #83616, #40508, #33432, #62336, #3632, #12612, #19240, #91176, #41457, #5517, #48097, #77001, #12130, #40976, #5037, #77951, #26813, #56655, #43348, #27759, #71312, #93073, #72245, #71790, #6442, #7817, #36707, #7360, #35787, #58503, #42401, #35317, #50453, #85504, #42877, #64242, #36242, #79355, #63760, #14017, #22048, #14490, #28227, #65160, #78413, #87348, #49975, #263, #28685, #14943, #57115, #20651, #740, #29146, #70843, #51370, #86414, #49521, #58042, #5976, #85955, #6912, #50917, #80261, #64700, #86894, #57571, #79801, #22497, #65628, #93526, #41932, #43798, #21107, #34849, #29625, #72698, #13552, #92590, #78867, #21570, #59906, #66083, #73175, #88748, #9203, #46130, #31019, #67469, #37175, #23894, #75033, #8294, #23441, #10146, #60825, #38081, #2130, #52309, #81186, #1195, #39012, #52763, #89668, #66992, #9685, #44264, #74084, #60366, #45182, #81644, #67926, #30533, #45645, #16791, #74554, #30076, #88286, #38567, #58961, #89204, #2598, #31478, #80725, #87809, #22958, #16332, #59435, #24356, #51832, #53231, #73635, #82113, #17272, #24837, #3050, #31934, #53720, #15878, #15397, #44734, #8746, #37623, #66534, #1653, #76890, #84440, #68862, #75487, #3991, #40399, #18194, #62222, #19588, #48457, #62717, #75947, #33803, #91547, #18659, #26703, #77358, #27166, #69317, #4445, #82587, #47046, #83984, #90587, #12018, #40868, #32410, #17734, #69786, #41344, #12492, #70278, #39946, #39470, #46589, #26225, #3518, #32866, #11077, #5411, #10612, #61755, #68387, #4917, #47987, #61308, #33325, #55592, #47526, #90144, #25294, #83501, #25748, #54172, #83041, #54629, #76431, #11552, #55119, #91051, #19132, #34276, #63183, #92014, #12985, #43242, #86776, #92475, #20999, #20545, #7256, #57465, #84908, #63653, #77837, #28575, #43689, #625, #35199, #27641, #64598, #7708, #50333, #57919, #42292, #48937, #71204, #13905, #85397, #35683, #21937, #50809, #36132, #49415, #65049, #152, #85846, #29032, #79694, #56054, #42758, #71675, #20056, #78305, #86308, #64127, #79240, #14382, #5867, #41823, #72140, #14836, #72586, #36592, #13444, #70734, #34737, #93423, #56540, #6331, #92962, #65506, #28121, #57010, #49864, #78763, #21460, #6809, #73966, #2480, #88157, #67804, #29511, #30418, #87691, #44144, #58392, #80599, #59309, #1532, #2002, #15756, #23316, #38441, #9080, #66867, #80147, #16668, #60245, #65971, #52189, #22844, #74425, #30895, #87237, #37062, #51256, #59788, #17143, #22384, #8629, #1082, #37960, #66415, #81070, #15287, #89083, #88629, #10025, #16215, #23776, #73048, #45066, #9554, #52641, #81521, #24232, #44616, #45523, #67350, #31357, #8178, #37506, #53109, #29962, #81987, #46009, #74914, #58848, #51711, #73520, #38895, #18073, #47397, #75369, #46926, #61184, #33208, #83864, #12369, #91428, #76308, #26582, #68268, #3872, #3390, #19017, #48338, #32278, #75828, #53595, #26099, #62101, #60706, #11434, #69666, #61639, #41217, #2928, #32751, #90022, #17615, #31813, #54049, #90472, #68741, #69202, #82919, #25629, #11900, #40285, #4331, #82468, #47869, #33677, #39349, #54511, #25175, #76772, #90934, #89546, #10483, #24709, #54988, #84320, #46466, #10952, #39818, #40749, #83383, #18531, #4798, #62586, #55471, #77239, #19471, #64485, #5290, #35085, #21349, #6216, #28005, #64943, #85275, #6696, #42644, #64004, #84789, #49294, #71561, #34160, #50220, #13792, #92842, #41705, #63063, #77716, #71084, #20425, #20883, #48809, #78189, #34624, #35571, #57356, #79590, #44, #49755, #28924, #70622, #56898, #5749, #86197, #21827, #63534, #50702, #93312, #72036, #56416, #91892, #13327, #85737, #92361, #78652, #7151, #36026, #79124, #27523, #14271, #43131, #28462, #57812, #86663, #14731, #70154, #27046, #55934, #42169, #19939, #12866, #66765, #1896, #87131, #43584, #30787, #2376, #9446, #31254, #977, #514, #81881, #80968, #58288, #87585, #36955, #67246, #7597, #22282, #22730, #65869, #60141, #36484, #58742, #29396, #59685, #8982, #65401, #88049, #16567, #8525, #72482, #51154, #44509, #8065, #80039, #15180, #29858, #73415, #15640, #16113, #51604, #37404, #52542, #23205, #44964, #44038, #88528, #74322, #72940, #66314, #80492, #23676, #73864, #1429, #30313, #59202, #37861, #88980, #52085, #81417, #45422, #38332, #24128, #53006, #9923, #76660, #54404, #91311, #39707, #11327, #45902, #75720, #61990, #46818, #68631, #11787, #32174, #47281, #83277 ),
 ( #17510, #33100, #62469, #46362, #26473, #40178, #18907, #3281, #38796, #61075, #3764, #75263, #90369, #47762, #40637, #90825, #10378, #25985, #54870, #10843, #83751, #69556, #55362, #32649, #61537, #17036, #39245, #18421, #25073, #69097, #4224, #60603, #74807, #4685, #33559, #67700, #2828, #68161, #31711, #89438, #76198, #24596, #25525, #53485, #82361, #89917, #53946, #82814, #17965, #70032, #77128, #63424, #21236, #34976, #41102, #48226, #63890, #78079, #50105, #6105, #42531, #12258, #92725, #79000, #5175, #92253, #14154, #35913, #13222, #70972, #34049, #49646, #71442, #13680, #77602, #86085, #19830, #85162, #62952, #55825, #34517, #78541, #91786, #84681, #43019, #6579, #71922, #48697, #12752, #27410, #7043, #42058, #41593, #64831, #93655, #28815, #26937, #56298, #84214, #19362, #70515, #5642, #20315, #49185, #27897, #35457, #56786, #85628, #64375, #93201, #20774, #28353, #57243, #36841, #7488, #10625, #79926, #72371, #59089, #43474, #87019, #15063, #87931, #87470, #22171, #23566, #53735, #23082, #51492, #75503, #58177, #51039, #66201, #36373, #58629, #43925, #51962, #1317, #79482, #29748, #37746, #30199, #72821, #80854, #391, #39483, #65759, #16001, #44396, #30664, #7946, #65286, #17748, #44853, #86542, #68405, #8416, #29280, #73756, #21712, #869, #22617, #66654, #3533, #80380, #8868, #73305, #1780, #57699, #46601, #50588, #15521, #37295, #59566, #88416, #82601, #14617, #92029, #69801, #13003, #55135, #26719, #61322, #91072, #77373, #62237, #83999, #27184, #47541, #62732, #4937, #26242, #47060, #11566, #33822, #90160, #12511, #91562, #19147, #4006, #25308, #39960, #33340, #76445, #76906, #11094, #40414, #90602, #55606, #19605, #41839, #56071, #12036, #84924, #32881, #48002, #61769, #48473, #77853, #25763, #70750, #84455, #34291, #18675, #54186, #69332, #40883, #54645, #41361, #63199, #20076, #70295, #83519, #5426, #48955, #32423, #83056, #18210, #75965, #68876, #4463, #5884, #6346, #21474, #21014, #14397, #43256, #20560, #34754, #7270, #14851, #50825, #43704, #92978, #85412, #63669, #50352, #78320, #49881, #28136, #72603, #27661, #85863, #49432, #36147, #72154, #56558, #57481, #86793, #6823, #92492, #13459, #86322, #42778, #57025, #42310, #35697, #79256, #65068, #29046, #64611, #167, #71219, #57939, #21952, #78779, #7725, #35219, #71694, #79709, #93437, #64145, #13920, #28591, #4296, #18496, #63031, #6185, #62553, #34127, #12335, #84757, #71053, #56380, #26550, #42135, #41673, #26064, #13297, #85246, #48778, #76275, #83348, #69634, #27486, #41181, #47360, #54479, #70121, #84290, #20393, #5258, #77684, #11401, #91862, #49264, #40253, #4762, #78159, #35052, #19440, #77205, #69169, #55905, #12835, #19905, #83830, #92331, #54953, #91395, #33176, #62065, #40716, #70591, #90899, #18984, #90439, #5718, #25596, #47836, #76738, #33643, #11865, #48306, #55438, #27016, #34593, #63502, #42611, #14240, #44480, #29827, #85707, #57324, #64911, #56865, #8495, #51123, #79558, #14, #80008, #72906, #20852, #6662, #50672, #43098, #13763, #15608, #86166, #78620, #65369, #49723, #93279, #21317, #479, #28892, #28431, #58710, #87552, #29367, #57781, #80460, #64453, #50188, #72450, #71528, #86628, #79088, #58259, #7569, #35538, #35992, #44008, #36454, #72003, #87102, #7122, #73385, #21798, #22252, #14699, #36927, #43554, #15148, #22700, #8030, #92810, #63969, #65841, #949, #51574, #27975, #37830, #38300, #46333, #23646, #88951, #66735, #17002, #68132, #3255, #17482, #30753, #82332, #75236, #67215, #10350, #32145, #75692, #24098, #52978, #37373, #1862, #38768, #45390, #60575, #89410, #80937, #66283, #24564, #89887, #61044, #25047, #88499, #88016, #1396, #74776, #52054, #81388, #59655, #53919, #30281, #52512, #23171, #53451, #2798, #59170, #81852, #39216, #2348, #16082, #44935, #31226, #16536, #73836, #8950, #74290, #60111, #9414, #9893, #45870, #67672, #82787, #31680, #17939, #46790, #91757, #41561, #47253, #69526, #69068, #55797, #12229, #39678, #18396, #32620, #77098, #92223, #49154, #83719, #76167, #19334, #47735, #76634, #3736, #70484, #48196, #85128, #33531, #5141, #68600, #4658, #84649, #40610, #62437, #5612, #25957, #41075, #70000, #91279, #25497, #18879, #34019, #61510, #19801, #62922, #26444, #11299, #90342, #40152, #11758, #54838, #55335, #83251, #84186, #4197, #26909, #48669, #20280, #34487, #77570, #63393, #33072, #12720, #61962, #27379, #56268, #90798, #10816, #54375, #79893, #64342, #70941, #22585, #65252, #93622, #14118, #357, #86985, #6072, #20743, #64798, #57210, #27862, #29716, #6544, #92692, #79447, #63859, #13647, #35422, #14583, #42982, #42499, #43891, #72788, #43440, #71887, #834, #78509, #71412, #86511, #56753, #78967, #93169, #72336, #21674, #34946, #50072, #58139, #50550, #28321, #7455, #49614, #58598, #86051, #36337, #28780, #51006, #21200, #85596, #36802, #29244, #13191, #87439, #57665, #7009, #22138, #42026, #35881, #15032, #7912, #78050, #65723, #88835, #67092, #45743, #32023, #17367, #81276, #3141, #2687, #80818, #68012, #46218, #9779, #37263, #44361, #30631, #82213, #2225, #8383, #15490, #31109, #45274, #75122, #59996, #38654, #73271, #23985, #10232, #66169, #59531, #39100, #60920, #74177, #38177, #1285, #16886, #67558, #74655, #44821, #53327, #15967, #52399, #30167, #23050, #1743, #31568, #59050, #51928, #89767, #60458, #51460, #73724, #8836, #88380, #80349, #9295, #37714, #87898, #66620, #23530, #16422, #52858, #81736, #89293, #24448, #16470, #24033, #16018, #82723, #10284, #10753, #81323, #52449, #67144, #39610, #74708, #88433, #46727, #75630, #61451, #1797, #2278, #3672, #17875, #44869, #45325, #52909, #8885, #23099, #39154, #38702, #81787, #68066, #32075, #37764, #59582, #9829, #31161, #66669, #68534, #74227, #30682, #53380, #23582, #9346, #60047, #82265, #16936, #88885, #32559, #51981, #17418, #45798, #80870, #67609, #2737, #31617, #60508, #89343, #46267, #75171, #3191, #60974, #89823, #24984, #53857, #90733, #62860, #33008, #13129, #4594, #19735, #77035, #63328, #76573, #40090, #49090, #91693, #25433, #6009, #41009, #4137, #26845, #54311, #25892, #91213, #5551, #34884, #62370, #33956, #12166, #84585, #70878, #56202, #26381, #41965, #41495, #54774, #90282, #85061, #48603, #76102, #83186, #69462, #27316, #69932, #47189, #18333, #5074, #84124, #20212, #55733, #77503, #11235, #12650, #77988, #69006, #33467, #61899, #83651, #19274, #70425, #18815, #34421, #92159, #47672, #11696, #40547, #55269, #48132, #85535, #35355, #14050, #29178, #27795, #64277, #80292, #93106, #28261, #72274, #49553, #64733, #57149, #58074, #7393, #20682, #35819, #43829, #36274, #85990, #65195, #6477, #15431, #71827, #86927, #50485, #36738, #50010, #13584, #22529, #298, #92624, #73206, #14524, #71346, #22080, #56688, #21140, #93560, #72730, #8325, #28718, #50950, #79387, #79833, #44298, #29657, #57603, #63795, #14973, #78903, #78448, #58537, #7851, #42436, #42913, #6946, #773, #43379, #86446, #21604, #65659, #87382, #51401, #52797, #89236, #58992, #16825, #67957, #1228, #45214, #3082, #82618, #31050, #23927, #30110, #2631, #24389, #60398, #30566, #39046, #66563, #38115, #87841, #8777, #81217, #31510, #22991, #37655, #31967, #53267, #24870, #1685, #59464, #16363, #53752, #88779, #88316, #60860, #89703, #75520, #15910, #74116, #17765, #46619, #51865, #23473 ),
 ( #52339, #67500, #17305, #37207, #66115, #81676, #45682, #80758, #9236, #38597, #67025, #82150, #46162, #44766, #73666, #75065, #2161, #59940, #74589, #9717, #10176, #48977, #48022, #25326, #54664, #4027, #34312, #68423, #25782, #61343, #33842, #69822, #3553, #55155, #77393, #69351, #10642, #39502, #11586, #68895, #54206, #32442, #61788, #40433, #76464, #76927, #90620, #4481, #19625, #84017, #12055, #90178, #91583, #41380, #47079, #33358, #32900, #55626, #40902, #83074, #18228, #75985, #4956, #92050, #11113, #83537, #39980, #19165, #47559, #62256, #18696, #70314, #62751, #84945, #91090, #26740, #26261, #84475, #48493, #12530, #5445, #63218, #27204, #56091, #20095, #71715, #92514, #57044, #50373, #13022, #57961, #21495, #6842, #49451, #70771, #85431, #78797, #92997, #28611, #56578, #28155, #42328, #14418, #65088, #87274, #72623, #57500, #7745, #78339, #13942, #13481, #188, #29548, #71239, #58428, #72173, #79729, #64165, #5904, #85882, #35716, #6368, #86344, #14871, #43725, #86815, #35239, #29069, #21973, #42799, #79277, #36628, #41858, #21034, #65550, #22420, #64630, #93456, #34774, #43275, #50846, #7289, #49902, #664, #36167, #77873, #63689, #27680, #20579, #16706, #15322, #51749, #17185, #38483, #38933, #15796, #80641, #1571, #67842, #9120, #22882, #74953, #10063, #89583, #29999, #30454, #31853, #46048, #73089, #44655, #52225, #44183, #51292, #67387, #66906, #81108, #2517, #60284, #8219, #87730, #37997, #59348, #1118, #2968, #73556, #66006, #52677, #37097, #8665, #37543, #81558, #16251, #66454, #60742, #80184, #45561, #45101, #58884, #88199, #23358, #59824, #74003, #2045, #30934, #74463, #88665, #23814, #9596, #31394, #89121, #24272, #53147, #82027, #41253, #32786, #47907, #11471, #91466, #10988, #68306, #77276, #90970, #53636, #34195, #69237, #32324, #26136, #82506, #25213, #25667, #33715, #63099, #90506, #62139, #40322, #19051, #5327, #84357, #54548, #70194, #69702, #54086, #24754, #19506, #76810, #10524, #17654, #3909, #55508, #4366, #75408, #46505, #33244, #18570, #48374, #55031, #11935, #39391, #83900, #3428, #61226, #40784, #90060, #4831, #82956, #18111, #83416, #62627, #46963, #47436, #26617, #12405, #75865, #39858, #68780, #76345, #61674, #43162, #27555, #14759, #57840, #50248, #77751, #84822, #71116, #28954, #42674, #48846, #55969, #71591, #85766, #86694, #13822, #79154, #19971, #6728, #21859, #12902, #6246, #50733, #43613, #20916, #78682, #41740, #57385, #14302, #21378, #85312, #76, #56450, #92877, #70653, #63569, #42202, #86228, #5781, #92395, #79617, #72063, #72509, #20460, #49328, #35115, #7629, #49785, #78222, #36514, #91927, #27082, #34655, #64035, #13361, #28039, #56928, #35600, #64515, #93341, #28492, #7180, #36055, #64973, #52569, #74353, #58316, #8097, #52115, #44541, #15210, #17065, #87614, #80067, #66794, #51180, #1008, #22765, #1924, #1457, #29888, #31286, #60172, #30818, #59233, #81913, #65896, #58772, #73893, #44067, #66343, #51635, #59715, #9010, #87160, #37434, #45453, #37889, #80521, #88558, #36984, #45932, #73444, #23706, #80998, #38362, #15674, #72968, #24157, #81449, #8554, #30343, #88079, #89010, #29426, #23235, #22309, #16597, #9476, #16140, #44992, #67276, #2406, #9953, #65429, #53037, #74840, #543, #67732, #89951, #68665, #10878, #11362, #25106, #3801, #47795, #83311, #76231, #89471, #26024, #69592, #75295, #32682, #3316, #83786, #40214, #2859, #46395, #60634, #69130, #26509, #77166, #18001, #10414, #47315, #75757, #39741, #31741, #4722, #4258, #19401, #61568, #33136, #24632, #90401, #18941, #25558, #54438, #33600, #53980, #62026, #90860, #18456, #53519, #46854, #54907, #82395, #76697, #11823, #40674, #39278, #17543, #68196, #62508, #82849, #91348, #32205, #55398, #61112, #84250, #48264, #38825, #7077, #85663, #35950, #77641, #13256, #12792, #28389, #57737, #41633, #86582, #6614, #14194, #92288, #5216, #27445, #63926, #70552, #20811, #43055, #71959, #86123, #5675, #57281, #21272, #42093, #50144, #64869, #50628, #92764, #27931, #12296, #34550, #13714, #20349, #35494, #64409, #55866, #41141, #93236, #93695, #28851, #21752, #63458, #62991, #70074, #34089, #56822, #79042, #91822, #49681, #26975, #84718, #49221, #19867, #48737, #6139, #78576, #56337, #71482, #85199, #78118, #71008, #35011, #42566, #81688, #7526, #52352, #31062, #46171, #43512, #81228, #46631, #67967, #68433, #45225, #16374, #59949, #3564, #38610, #74129, #10656, #39512, #25337, #59478, #88789, #61355, #75531, #36411, #9248, #16837, #72410, #79518, #3093, #2643, #45693, #31977, #89715, #65326, #23485, #67513, #23937, #29319, #32455, #38126, #431, #82161, #88332, #67038, #2176, #17319, #74602, #52809, #90189, #14656, #75075, #9732, #31521, #60409, #89248, #24400, #53278, #10186, #39055, #60870, #24881, #53762, #82628, #17777, #62765, #54677, #26754, #90634, #70784, #62271, #77407, #40915, #27219, #40446, #4041, #13036, #55638, #83086, #63704, #4970, #61802, #84492, #18240, #83550, #55169, #63233, #92529, #26274, #91598, #69836, #48506, #34789, #20111, #84031, #5919, #5458, #18709, #54217, #48991, #12544, #39992, #47092, #33372, #84960, #33855, #11127, #75997, #19638, #48036, #76940, #77892, #41394, #70328, #68910, #34326, #41873, #32912, #91106, #25796, #47573, #12068, #92064, #76478, #56105, #11600, #69363, #4494, #19176, #57061, #28626, #49465, #93013, #71730, #86832, #85446, #28171, #87291, #14887, #15341, #85897, #21050, #6857, #44202, #79294, #49917, #51310, #80202, #66024, #6384, #35732, #8236, #22437, #78354, #78813, #57516, #20595, #27695, #43741, #43292, #86360, #72641, #36647, #13495, #64180, #14435, #64645, #71255, #73109, #13959, #42344, #29087, #35255, #42816, #93473, #57979, #21512, #50390, #37115, #56592, #21990, #72189, #7305, #36185, #65104, #205, #50863, #79745, #7761, #65567, #681, #29565, #58446, #74972, #9617, #1590, #67408, #37562, #17673, #9139, #24292, #81579, #67863, #81126, #44673, #53656, #2537, #30017, #10546, #45580, #8684, #31416, #58901, #30472, #2064, #10084, #39411, #66926, #38504, #16727, #89142, #75427, #60762, #30955, #46526, #46066, #59368, #1136, #89603, #53168, #80660, #87747, #74022, #31873, #74485, #51770, #22899, #60304, #82048, #88220, #17205, #66473, #15816, #38016, #38952, #2987, #24773, #16270, #73575, #82525, #23376, #52245, #45120, #59843, #88684, #23832, #52697, #68800, #69257, #77295, #77772, #40340, #11955, #83920, #62649, #48869, #34213, #4385, #19990, #19525, #3929, #84842, #63119, #26638, #54106, #61245, #47458, #5347, #19072, #25232, #32346, #47926, #62160, #91948, #76829, #55528, #90080, #40804, #27102, #82978, #76365, #55987, #12920, #90989, #55051, #18129, #33736, #84377, #91485, #61693, #70213, #32803, #33263, #46983, #39879, #18592, #48392, #75883, #90524, #68327, #12425, #3451, #25686, #54567, #11491, #11009, #26159, #83437, #69721, #4852, #41276, #20480, #85784, #22327, #7647, #63589, #35133, #42693, #34674, #80085, #28973, #57403, #71612, #57858, #50751, #92413, #78242, #28510, #20935, #85330, #87178, #64056, #56471, #43180, #27573, #71136, #92898, #72082, #6746, #6265, #36532, #65447, #7198, #35619, #58336, #42221, #28057, #50266, #49347, #64534, #56947, #36073, #79175, #13379, #13842, #21879, #49803, #93359, #78700, #64990, #14320, #86244, #21395, #79635, #94, #86714, #14777, #43630 ),
 ( #563, #29448, #51198, #72527, #41761, #70672, #5801, #29906, #59250, #8573, #38842, #72987, #30361, #65916, #38382, #74370, #8117, #59733, #81930, #73911, #53539, #15228, #16158, #73461, #58790, #44084, #66360, #45010, #81014, #81467, #1475, #9027, #24175, #88575, #52586, #1028, #2423, #45952, #51653, #37906, #37451, #60189, #16615, #37003, #22784, #87634, #45470, #2875, #80539, #88096, #15696, #23723, #52134, #66811, #44558, #74858, #9494, #89489, #1941, #67294, #23256, #30838, #89027, #31303, #53055, #9970, #17083, #67749, #31759, #60652, #24650, #61585, #54924, #17560, #62525, #26040, #11380, #53997, #75313, #89969, #83327, #3818, #33152, #61132, #32699, #46871, #18959, #69608, #91838, #77182, #4738, #26992, #12312, #62042, #41156, #82866, #18473, #18019, #33618, #34105, #75775, #63007, #76713, #84267, #68686, #10431, #90417, #40231, #10895, #90877, #19417, #48280, #91367, #39760, #26526, #55415, #47333, #70091, #5233, #82413, #69146, #4274, #46412, #25574, #83805, #54455, #11839, #40690, #32223, #39295, #68214, #3334, #25123, #76251, #47812, #12810, #450, #93252, #70567, #6156, #49239, #79533, #19882, #71025, #41650, #79059, #21288, #48753, #6631, #28865, #20827, #55881, #84733, #56839, #20368, #5692, #77658, #13272, #85680, #27949, #28406, #42109, #49696, #64885, #35511, #57297, #34567, #43071, #86599, #92304, #78592, #78134, #7094, #86139, #63475, #27461, #56353, #50162, #43528, #85215, #35028, #63942, #64426, #92780, #13733, #42584, #21768, #14210, #36426, #71499, #71975, #35965, #93710, #57753, #50644, #14672, #72425, #7542, #65343, #1833, #23137, #43978, #8466, #30719, #58229, #9384, #66704, #52019, #920, #22222, #36893, #30250, #44448, #73806, #8001, #73354, #87525, #59619, #59141, #22671, #72877, #87073, #80433, #87984, #1368, #88468, #15578, #80905, #38267, #8920, #23615, #79980, #16506, #60081, #65809, #16051, #51543, #74261, #52482, #51091, #29799, #15117, #81356, #16971, #67641, #37346, #58680, #37798, #66252, #44903, #45358, #88918, #67179, #9861, #2314, #31196, #24068, #52944, #81821, #45836, #74741, #38736, #29334, #33040, #69038, #90312, #17450, #75660, #4167, #31649, #76604, #40121, #25464, #68098, #89377, #10318, #3705, #17907, #47224, #75204, #46760, #61010, #61929, #83686, #12197, #91248, #76134, #26412, #3223, #32591, #32113, #18847, #48164, #89856, #77066, #90767, #4625, #82754, #24533, #10784, #54345, #25016, #11268, #33499, #62406, #11728, #53888, #47705, #40580, #61481, #69495, #55302, #41039, #83219, #18364, #2767, #39645, #25925, #68569, #54808, #84155, #46299, #60539, #19303, #53416, #82299, #39186, #27346, #26877, #14551, #13613, #84618, #20243, #63359, #93589, #33986, #85095, #55764, #93132, #35388, #62889, #20711, #42948, #34912, #69968, #5108, #28288, #56717, #71854, #56232, #19766, #28748, #42466, #91725, #79417, #49581, #77536, #71376, #48635, #70453, #70906, #78932, #12687, #41993, #6510, #85564, #64308, #50518, #35847, #6040, #21640, #21168, #5580, #86474, #64765, #57178, #41527, #34451, #49121, #6975, #78476, #92190, #78017, #86018, #63824, #57631, #50037, #14083, #13157, #92657, #27829, #7423, #51428, #74145, #88802, #37234, #30136, #36304, #8802, #30593, #66589, #36769, #45239, #72757, #44329, #65220, #15000, #87407, #37682, #325, #43860, #9262, #59497, #31075, #7878, #65689, #22554, #59963, #1255, #803, #67055, #2191, #81701, #22108, #80318, #23949, #38139, #29210, #29683, #73240, #58109, #43408, #88348, #59020, #8351, #23499, #52367, #86955, #79862, #87867, #15457, #50977, #52821, #58567, #66139, #44791, #23017, #51895, #80788, #73692, #15937, #1710, #72302, #81242, #16389, #10669, #33385, #17333, #46183, #25348, #2654, #17790, #75089, #76011, #54229, #38621, #82640, #90647, #83097, #10198, #18251, #53291, #62284, #24894, #55185, #47104, #31533, #60881, #39067, #40458, #74618, #31989, #67524, #40006, #11144, #9746, #61367, #83563, #75544, #16850, #45705, #46643, #67980, #60420, #89260, #3106, #39524, #68445, #68923, #89732, #3580, #25809, #90200, #4054, #24411, #32924, #47586, #82177, #32469, #53774, #61814, #54689, #18725, #76490, #11613, #69376, #4506, #91120, #26291, #35153, #14337, #71629, #6761, #78259, #43646, #43196, #29462, #28528, #65007, #20497, #93377, #86730, #64553, #57421, #7663, #78716, #7214, #72097, #86261, #42240, #42712, #36087, #49365, #21893, #108, #21412, #92913, #13396, #64074, #35635, #13857, #50287, #6282, #79194, #85800, #28987, #57875, #58351, #36546, #50766, #72542, #28075, #79650, #56963, #14791, #87191, #20951, #85349, #65462, #579, #71153, #49819, #62485, #34066, #10501, #55844, #13237, #42073, #56316, #68286, #27426, #85181, #12275, #20330, #70989, #20791, #62968, #91802, #74933, #39370, #77619, #84229, #5656, #34531, #24733, #10043, #63439, #34991, #6121, #63908, #33576, #31833, #48243, #19845, #26954, #70532, #56801, #92743, #41119, #27914, #49200, #4699, #85643, #38913, #92269, #60724, #67822, #55377, #2947, #84698, #89563, #53616, #48716, #70051, #82486, #12768, #78096, #17634, #41610, #46485, #75388, #19378, #91325, #26487, #5193, #77145, #13695, #15080, #36858, #72837, #43036, #51507, #79020, #50607, #71462, #21252, #93674, #43940, #42547, #50122, #15540, #65774, #37310, #14173, #71938, #28832, #66217, #7505, #7059, #73320, #8431, #87947, #28368, #57716, #30214, #44412, #6595, #35929, #79498, #35473, #49662, #883, #65303, #14634, #29764, #58643, #64390, #86103, #36390, #86562, #93216, #1332, #64847, #57260, #51054, #21731, #43492, #72388, #79942, #410, #29297, #59105, #78557, #7964, #58192, #87035, #22186, #87485, #22635, #80395, #44482, #80462, #37375, #8497, #22702, #73387, #30284, #66285, #15610, #1398, #59172, #51576, #26177, #41294, #4871, #84859, #4402, #61709, #70688, #84394, #46999, #27594, #62666, #25701, #19542, #75902, #18610, #19089, #27121, #56491, #11027, #91965, #55544, #40820, #83455, #39895, #54583, #47943, #33281, #91499, #90543, #62176, #76381, #48408, #5364, #18145, #12939, #26655, #41778, #47474, #76845, #11509, #34230, #63606, #40356, #92430, #12446, #20011, #91008, #68816, #55067, #69739, #69273, #77311, #48889, #77790, #56004, #83936, #63136, #5818, #11972, #34692, #3947, #32819, #33754, #70229, #85350, #49820, #86731, #93378, #14792, #43647, #35154, #20498, #72543, #44098, #51211, #73004, #42713, #42241, #29920, #28988, #6283, #35636, #78717, #15241, #49366, #6762, #71154, #7664, #50767, #78260, #36088, #58352, #50288, #13397, #64075, #86262, #13858, #92914, #28076, #71630, #21413, #57422, #57876, #64554, #79195, #580, #65008, #21894, #56964, #36547, #22340, #85801, #14338, #28529, #65463, #79651, #20952, #43197, #72098, #29463, #8132, #7215, #109, #87192, #80102, #37015, #65929, #1041, #24665, #2435, #39307, #81478, #53066, #87648, #23734, #9981, #88586, #16627, #53552, #73922, #89038, #31314, #52597, #73474, #37917, #60200, #37464, #9039, #23270, #24188, #45965, #68224, #82424, #38397, #17574, #30374, #59745, #59265, #74871, #10441, #88113, #3344, #81941, #60663, #45022, #51666, #66821, #45481, #52146, #67306, #89500, #46423, #38853, #81026, #67760, #2886, #74380, #31771, #75325, #58804, #9508, #17098, #22799, #16170, #80556, #1959, #15710, #44571, #8586, #66373, #1490, #30852, #91850, #19893, #83337, #82876, #70579, #69622 ),
 ( #41167, #76726, #4750, #18029, #19429, #63018, #68698, #90889, #90428, #77194, #33630, #61144, #39773, #54009, #62540, #48764, #32235, #11390, #3828, #40702, #69158, #4285, #25133, #27004, #91382, #12823, #54939, #26538, #89979, #26052, #12323, #62054, #83819, #55892, #47346, #55425, #84278, #18971, #46883, #40242, #48292, #75785, #70106, #5246, #47824, #32710, #10905, #61595, #33163, #76263, #11853, #84746, #25584, #34116, #77670, #41662, #54467, #18483, #63489, #64900, #86615, #28881, #92796, #7557, #35042, #6648, #27475, #71039, #49711, #1, #92320, #6173, #65357, #21785, #87088, #63956, #27964, #78606, #22237, #57312, #56853, #29353, #58245, #43994, #78147, #13751, #79994, #464, #56367, #85694, #35528, #85231, #5704, #50661, #21305, #64441, #79547, #14687, #20382, #42122, #86154, #42599, #49252, #51108, #20840, #13285, #7109, #71514, #93267, #28421, #35980, #50178, #79074, #15131, #34580, #57769, #14226, #43087, #71991, #43542, #72439, #36442, #73822, #8481, #38283, #81373, #934, #44920, #52960, #16522, #73369, #45373, #15591, #89394, #80923, #2332, #59637, #45852, #59156, #22685, #31664, #74276, #8015, #82316, #23631, #80446, #9399, #36909, #37360, #8935, #81837, #17466, #37813, #67196, #88484, #31211, #53432, #38753, #66720, #24548, #24084, #66267, #72891, #67657, #60096, #58694, #65827, #52037, #9877, #52496, #29813, #87538, #88935, #1848, #2783, #16987, #74758, #51558, #60556, #44464, #30735, #1382, #30264, #88000, #23153, #16066, #90782, #25032, #61495, #10800, #76620, #33516, #55780, #41058, #25942, #69984, #17923, #47238, #46774, #62422, #91741, #75675, #84633, #40596, #48180, #32606, #39201, #90327, #4182, #39662, #54823, #77081, #12212, #26427, #68584, #91263, #55320, #76150, #84170, #5124, #46316, #33056, #61945, #75220, #3720, #47720, #54360, #69510, #4641, #89871, #10334, #19318, #34001, #62905, #68113, #25481, #3239, #32129, #83701, #61025, #83234, #18381, #53903, #82771, #11283, #40137, #69053, #11743, #18863, #64323, #86494, #78492, #58123, #19782, #20726, #78033, #34469, #48653, #70924, #49596, #85579, #86034, #6055, #13630, #28763, #93149, #57193, #70467, #6991, #50533, #56250, #42481, #13173, #64780, #21183, #77554, #27361, #41543, #50054, #7439, #12703, #92674, #85110, #28303, #56733, #71394, #5595, #79431, #78950, #341, #6527, #14100, #63375, #35403, #93605, #42964, #71869, #14567, #34927, #35863, #57646, #21657, #92205, #27844, #43423, #20260, #72318, #36321, #49136, #65235, #42008, #63842, #29228, #2206, #2668, #59032, #30610, #8815, #81257, #67539, #52839, #23031, #38636, #38157, #22568, #9761, #81716, #45254, #72771, #79875, #66151, #23965, #37695, #43874, #50990, #66601, #80801, #16865, #1723, #74158, #15015, #59512, #45724, #7896, #1267, #74634, #31547, #15949, #73705, #36785, #52380, #9274, #16402, #80330, #88817, #51442, #87879, #65705, #58581, #37247, #67072, #817, #87420, #86968, #31090, #22122, #15473, #44344, #30149, #29698, #44804, #73254, #8366, #51910, #88361, #23511, #59978, #40943, #55201, #82193, #53786, #61381, #53308, #5001, #47601, #76031, #90214, #76504, #69390, #17347, #3123, #47118, #39540, #10213, #12096, #82654, #75103, #61830, #46198, #89749, #17803, #90663, #25363, #24909, #84056, #19204, #25823, #54243, #76967, #60901, #46656, #68937, #39081, #83113, #75560, #54703, #4068, #67995, #32484, #40473, #32938, #10682, #83580, #32003, #69863, #68462, #18743, #11160, #33399, #3597, #18264, #48063, #11627, #89275, #60439, #4523, #24426, #40021, #62298, #91139, #22810, #93388, #63260, #79205, #51679, #86742, #5483, #58816, #87660, #73486, #12578, #14348, #15722, #1052, #55667, #28541, #36099, #26780, #33884, #22351, #50777, #65019, #51224, #44112, #84518, #70357, #21904, #43207, #77434, #80568, #57432, #48533, #36560, #19665, #86273, #21425, #65475, #119, #50299, #29931, #44583, #593, #29000, #62792, #34355, #72109, #43659, #41425, #57886, #7225, #29475, #72554, #79663, #14804, #15252, #7676, #58363, #87203, #80113, #91627, #73015, #8144, #37027, #65941, #88597, #52156, #61156, #74883, #37475, #18044, #53078, #16182, #9993, #66385, #9050, #9522, #17586, #46896, #74393, #45977, #24201, #2899, #82888, #68238, #38409, #54021, #53564, #37928, #25146, #3360, #60676, #88124, #1501, #81491, #39320, #81955, #59278, #30386, #17112, #2448, #32249, #38866, #89515, #23282, #67772, #89991, #81038, #16638, #8598, #45034, #31326, #89052, #73935, #31782, #24679, #82437, #1971, #10454, #66835, #67318, #30863, #59757, #52609, #23746, #46435, #45492, #60213, #75338, #10921, #40720, #27019, #11868, #33647, #70594, #90902, #12338, #48309, #69637, #90442, #54956, #77209, #39788, #55908, #19443, #4765, #47363, #68711, #83351, #76741, #26068, #26553, #54482, #83833, #40256, #41185, #63034, #85249, #5721, #55441, #34596, #76278, #62556, #11404, #91865, #27489, #69172, #56385, #70124, #77687, #62068, #3841, #18987, #91398, #4300, #84293, #12838, #41676, #84760, #33179, #19909, #48781, #5261, #63506, #92334, #20396, #34130, #75797, #32723, #47839, #61609, #25599, #18500, #7571, #92814, #49267, #36456, #8033, #15150, #36929, #6665, #6188, #87555, #86632, #63974, #93282, #42614, #72908, #13300, #64456, #35055, #72452, #14702, #42138, #17, #22254, #14243, #78162, #71056, #50191, #13766, #27978, #56868, #35542, #79093, #21320, #21800, #28434, #43101, #58261, #28895, #50674, #85710, #65371, #80010, #20855, #72007, #71532, #482, #79560, #49726, #78623, #57327, #43556, #65843, #86169, #7125, #35995, #57784, #64914, #29369, #87104, #51126, #44010, #951, #29829, #58712, #68261, #48329, #39811, #54980, #18524, #4788, #18066, #75361, #84312, #4324, #60699, #41208, #76300, #39342, #33201, #89538, #32271, #32743, #40741, #70146, #3864, #69194, #47390, #26091, #12360, #91420, #61632, #77231, #76764, #61177, #31806, #26573, #83856, #17608, #24702, #10945, #62578, #11426, #82460, #53586, #40278, #25622, #55462, #62092, #19008, #46459, #90925, #19463, #10476, #68733, #3383, #90013, #54504, #47861, #25168, #11891, #69658, #33668, #54042, #82912, #46919, #90465, #75821, #83375, #49285, #64476, #63056, #5741, #64935, #86189, #86654, #63526, #34615, #78181, #21819, #56889, #70614, #28916, #57804, #43576, #77709, #13319, #79579, #36, #27039, #92353, #6208, #91885, #5282, #21341, #20875, #35076, #50211, #14263, #55928, #41696, #85729, #42159, #48799, #50694, #27511, #19931, #6686, #84780, #56407, #85268, #35563, #63993, #20417, #14723, #34151, #93304, #92834, #12858, #71076, #27997, #13784, #49747, #78644, #42635, #28454, #71551, #57349, #79115, #43121, #72027, #7143, #36017, #37851, #36476, #72929, #38325, #59677, #60134, #36948, #8056, #22721, #88973, #30305, #44029, #2369, #31247, #17025, #51146, #51596, #53000, #67239, #505, #65861, #73407, #65392, #72474, #88520, #88039, #8517, #23668, #81409, #29387, #15171, #59193, #80482, #22272, #24121, #969, #87122, #73856, #58280, #29849, #58732, #8973, #37396, #87577, #81874, #7590, #66757, #66305, #80030, #15632, #44501, #80960, #1419, #23196, #52077, #1885, #16104, #44956, #30778, #52534, #16559, #45413, #74312, #9438, #62458, #53938, #69087, #32639, #18898, #32166, #89431, #4676, #18413, #74799, #55353, #90360, #53475, #47273, #9916, #46355, #46811, #54859, #84205, #17958, #83269, #61529 ),
 ( #38789, #82807, #76651, #91301, #39698, #25517, #67693, #11319, #33090, #4215, #39238, #47753, #75713, #10836, #76189, #3274, #68623, #83741, #54396, #40170, #2821, #61981, #11776, #82354, #3757, #10371, #90816, #25975, #31703, #17502, #60596, #40628, #33550, #45894, #25066, #75256, #69546, #26464, #24587, #68154, #61067, #89908, #93646, #42048, #13671, #48214, #78069, #64366, #49175, #70962, #14145, #34507, #49637, #85619, #13212, #34039, #92243, #20765, #77118, #93192, #56777, #6095, #84669, #12247, #26927, #20304, #63414, #63879, #91776, #27398, #77590, #78532, #6568, #28806, #43009, #92717, #71913, #19820, #34967, #48686, #35447, #64822, #12741, #57690, #42521, #21227, #5632, #41093, #56288, #27887, #41583, #71433, #50096, #78990, #28344, #70505, #57234, #86076, #7034, #35904, #19352, #70021, #5164, #62942, #55815, #85151, #87923, #859, #15993, #44845, #36364, #86533, #73748, #45299, #52426, #74204, #43917, #43465, #31136, #30191, #7479, #36831, #79918, #16447, #50578, #7937, #72362, #8860, #51953, #79473, #37286, #59557, #51484, #21701, #14607, #87462, #51030, #65277, #382, #72812, #65750, #23074, #59080, #80372, #29270, #29740, #80844, #58166, #66646, #37738, #15513, #87010, #22162, #15055, #22609, #58621, #66193, #44386, #73296, #8408, #1772, #30656, #2253, #81301, #1309, #9321, #88407, #23557, #38204, #67118, #11670, #89319, #40519, #54285, #61873, #46243, #52882, #75147, #17850, #24474, #39583, #90704, #25865, #40062, #53353, #11204, #68980, #89793, #4110, #54746, #4567, #46701, #75603, #60022, #82238, #61425, #68039, #83155, #18307, #9804, #88860, #47164, #18786, #83624, #47645, #17394, #16912, #24009, #3641, #74680, #10259, #39127, #76547, #81762, #3165, #45770, #76073, #25406, #38678, #10727, #32982, #24957, #67583, #2711, #60944, #32050, #31593, #60482, #53833, #82699, #68506, #32532, #90257, #69437, #42409, #77960, #70852, #84100, #20657, #64251, #69906, #92133, #91668, #78421, #34856, #62344, #40985, #55243, #5984, #21114, #71798, #12620, #5045, #41940, #70397, #5525, #26352, #93080, #63769, #14024, #56175, #27768, #91184, #27288, #13559, #63302, #85033, #28234, #77011, #78876, #55708, #48107, #92598, #19249, #62835, #84559, #56662, #20183, #26821, #57122, #85963, #85511, #49063, #49982, #33926, #19706, #49527, #12139, #34395, #48577, #71320, #6450, #77477, #13102, #35325, #42885, #41466, #33441, #43356, #23449, #14951, #30086, #87357, #73644, #86902, #50460, #59443, #73183, #35794, #16340, #51378, #14499, #8302, #64707, #7369, #7826, #15886, #45190, #72706, #44273, #22507, #1204, #81194, #66541, #36716, #52317, #51840, #36250, #6920, #1662, #58970, #86423, #93534, #79810, #37633, #80269, #57578, #28692, #15407, #749, #30543, #37184, #87817, #21578, #66091, #88294, #79363, #43806, #72252, #65168, #29633, #22968, #274, #80733, #44742, #8754, #29154, #58051, #22057, #65636, #50926, #58512, #24364, #39476, #38092, #74564, #39953, #61315, #61762, #38574, #9693, #53242, #90595, #31943, #45656, #3999, #32874, #18668, #52773, #82124, #54636, #68869, #2138, #67477, #75041, #67002, #74093, #90153, #89678, #10153, #25301, #83049, #31027, #16800, #60834, #17281, #39020, #18201, #83510, #46138, #17741, #24845, #68396, #9212, #25755, #67935, #59914, #54179, #2606, #88756, #23902, #32416, #81652, #31486, #3058, #11087, #53728, #60374, #89213, #82594, #46595, #75494, #10618, #47053, #3526, #75956, #78313, #11559, #55599, #13452, #92971, #41353, #34283, #40407, #12993, #34746, #70742, #40875, #49423, #76898, #48465, #69325, #19139, #91554, #41831, #4454, #47994, #42303, #63661, #35210, #12028, #69793, #26711, #64138, #5418, #4926, #71212, #6339, #85854, #26234, #84447, #28129, #57018, #33332, #33812, #77365, #62229, #47534, #92484, #63191, #12501, #27651, #56550, #91060, #83992, #92021, #19597, #55127, #76438, #62724, #70285, #48947, #27176, #56063, #84916, #77845, #20066, #5876, #85405, #20553, #80158, #14845, #37514, #21468, #50344, #29521, #6817, #21946, #79250, #15296, #58401, #42768, #86787, #1091, #87247, #14391, #22393, #57475, #66424, #29040, #44153, #7717, #87702, #7264, #64605, #73528, #51265, #49874, #30426, #65518, #28583, #73060, #78772, #43250, #8637, #59317, #161, #86316, #8190, #57931, #50819, #13913, #80609, #37071, #1543, #43698, #65980, #71687, #79703, #29972, #72597, #36601, #15767, #36141, #58856, #22853, #637, #35691, #51719, #44626, #93431, #21007, #72148, #65060, #59796, #81079, #2013, #89091, #9564, #38903, #66876, #38452, #52649, #24721, #75378, #5182, #84220, #67812, #19367, #88637, #24243, #23785, #10491, #41108, #81529, #70040, #82476, #90031, #74433, #16223, #67358, #46019, #16677, #2937, #25183, #55368, #68276, #45532, #39360, #3398, #53117, #32289, #48232, #34056, #74922, #10033, #88168, #2488, #89553, #31365, #17623, #46474, #37968, #23327, #61194, #77135, #12266, #52197, #60254, #45074, #73974, #31823, #9091, #81997, #17153, #30906, #60714, #53605, #19835, #86092, #28358, #26943, #13684, #35919, #27903, #7494, #62958, #63895, #27415, #77607, #91792, #20320, #92731, #34981, #35462, #49190, #56791, #71928, #42536, #6584, #48703, #50111, #93662, #5647, #85633, #56303, #14161, #64381, #55831, #70521, #84686, #93206, #21242, #12758, #41599, #79006, #21719, #28822, #50594, #78085, #34522, #63429, #57250, #92258, #13228, #85169, #86548, #42063, #70977, #6110, #43025, #7050, #20780, #71447, #64837, #49652, #78546, #57705, #79488, #14623, #43481, #72377, #87474, #66205, #8420, #8872, #22622, #1321, #45310, #80858, #73760, #87024, #23570, #67132, #72826, #30203, #873, #81312, #37750, #65292, #43929, #58182, #66658, #24021, #74695, #15526, #7951, #44857, #73309, #37299, #29286, #2266, #1785, #16924, #59094, #30668, #396, #87935, #16458, #23086, #51968, #31149, #51496, #59571, #88421, #16005, #51043, #44401, #52437, #22175, #74215, #9334, #38217, #36846, #79931, #65763, #60035, #80384, #88872, #15067, #52895, #29752, #81774, #45783, #36379, #58633, #83172, #4580, #75159, #10741, #10272, #25880, #55257, #39141, #84112, #4125, #11684, #89810, #2725, #24972, #61440, #68052, #18322, #40535, #69450, #83638, #3179, #54761, #18802, #39598, #47660, #33455, #48120, #90270, #25421, #9817, #32063, #11222, #17863, #32996, #61887, #31605, #47178, #62358, #67597, #46715, #91199, #19262, #3658, #54299, #60494, #68994, #90719, #76561, #60958, #26368, #53846, #68521, #89331, #82712, #75617, #38690, #24486, #32547, #53366, #82252, #17407, #76088, #40077, #46255, #93548, #34870, #48591, #6934, #35807, #21594, #55721, #27302, #57591, #42900, #5060, #70413, #77976, #69920, #77024, #64266, #92613, #13117, #93095, #85978, #33943, #19721, #63783, #56190, #26833, #28706, #5538, #91682, #78437, #62848, #12636, #34409, #13573, #41953, #41483, #71814, #64721, #42423, #70866, #86435, #77491, #63316, #85525, #84573, #5997, #92147, #71335, #20671, #85049, #49077, #57137, #49542, #20198, #6465, #27783, #12152, #56677, #35342, #28249, #49996, #21128, #78891, #40997, #14038, #79377, #59931, #1216, #58063, #51855, #14514, #50940, #51390, #59455, #88770, #22519, #87830, #66105, #44756, #31041, #16353, #80281, #2151, #1675, #79822, #67016, #45204, #8767, #36264, #43369, #29647, #81208, #30100, #7383, #72265, #58982, #44288, #74106, #22981, #65648, #14963 ),
 ( #30557, #88306, #15420, #23464, #9226, #50474, #8315, #80747, #65184, #43819, #15899, #58526, #73656, #37645, #287, #29168, #66554, #38106, #86917, #22070, #7841, #72718, #36728, #52330, #762, #87371, #73195, #37197, #81667, #39036, #74579, #47069, #83065, #16814, #68414, #90611, #82609, #62246, #23917, #24860, #82140, #38588, #52788, #75056, #53743, #89693, #90169, #10167, #17756, #32891, #3544, #61332, #9707, #11104, #54654, #60389, #46609, #17296, #68885, #25317, #45673, #31500, #67491, #54196, #11575, #2622, #3073, #89227, #32432, #60851, #75511, #24379, #83528, #18219, #4472, #10633, #75976, #53257, #39492, #4016, #39970, #61778, #18687, #67949, #25772, #47550, #76455, #46152, #31957, #40424, #69341, #33349, #34765, #20086, #62742, #84008, #4947, #92040, #12521, #41849, #69811, #19156, #63209, #71230, #5894, #91574, #63679, #33833, #13931, #5436, #20570, #77863, #64155, #77383, #40893, #49893, #92503, #26252, #6833, #70762, #26730, #27671, #55146, #55617, #27194, #6356, #35707, #56082, #56569, #13013, #85422, #71706, #57035, #84934, #42789, #42320, #84465, #91081, #85873, #49442, #76917, #48012, #70305, #28146, #78330, #12046, #19616, #13471, #48967, #21024, #35230, #92988, #48484, #78789, #41371, #34303, #72614, #1560, #16240, #58417, #51281, #28601, #29989, #51735, #87719, #57951, #66441, #178, #65539, #86334, #36157, #14862, #58872, #57491, #65079, #30443, #80628, #52214, #29059, #86806, #43715, #81097, #22409, #21963, #88187, #23346, #9109, #43266, #7736, #45090, #59335, #21484, #50837, #654, #50364, #64621, #15784, #80174, #29538, #44643, #73544, #79267, #7280, #15312, #36617, #14408, #73991, #79720, #72164, #65996, #87264, #44171, #73078, #1107, #8209, #37087, #93447, #22870, #8653, #37530, #54074, #45550, #74450, #2956, #88654, #53134, #9583, #24742, #31841, #60272, #81546, #60731, #89108, #24260, #2033, #32310, #89570, #82944, #46036, #53624, #66893, #17172, #75396, #82015, #74941, #61213, #2504, #82494, #17642, #10051, #23803, #38921, #46493, #37985, #68294, #10509, #67830, #38471, #52666, #67375, #39379, #3415, #90048, #31382, #25200, #18096, #46950, #30923, #59813, #16694, #8501, #23650, #487, #29833, #29374, #44939, #74295, #58265, #9419, #23177, #30758, #15155, #21805, #44014, #80466, #87108, #37379, #59660, #88503, #8955, #22258, #73840, #37834, #58716, #66740, #52516, #67221, #15615, #44487, #28899, #51131, #30289, #36933, #52060, #80942, #72457, #57787, #16087, #81392, #16540, #45396, #80014, #79564, #86637, #66290, #43560, #72912, #8038, #38306, #50678, #65847, #14707, #1866, #88021, #7575, #73391, #36460, #87560, #65375, #955, #22706, #51580, #1402, #59176, #53456, #32148, #68137, #68605, #82337, #61049, #11304, #46794, #39681, #52983, #83255, #33076, #38772, #89892, #60579, #47258, #3742, #31230, #9898, #24102, #32624, #83724, #40614, #3258, #76172, #10821, #2802, #61514, #67676, #18884, #10354, #25501, #82791, #69073, #17485, #45875, #54842, #90346, #60116, #11762, #75696, #31685, #54379, #88955, #89414, #25050, #40156, #2353, #53923, #18399, #17943, #4201, #76637, #61965, #90802, #47739, #25961, #24568, #81857, #17006, #74781, #46337, #75239, #39219, #6549, #20288, #26450, #33536, #49162, #63399, #35428, #85133, #27868, #91284, #78055, #64350, #62441, #77574, #93176, #21208, #92228, #56274, #55339, #34952, #56761, #92698, #62928, #71417, #5147, #70490, #84190, #41080, #19805, #63864, #19338, #70004, #28328, #85602, #57218, #34024, #91762, #48673, #86058, #27384, #26914, #50078, #78973, #14125, #48201, #12725, #69530, #4663, #77102, #55801, #5618, #12233, #84653, #20749, #13196, #34493, #49620, #78516, #41568, #42032, #70946, #6078, #13653, #42505, #65259, #57673, #44368, #21681, #72344, #365, #73279, #72795, #7462, #8844, #37722, #8392, #36810, #59539, #43447, #36345, #51467, #50558, #43898, #29251, #37270, #80356, #64805, #42990, #30175, #1753, #66628, #30640, #58147, #93629, #81285, #15497, #79455, #86993, #22145, #88389, #7016, #51013, #14590, #66176, #1293, #79900, #87446, #15977, #7919, #71896, #15038, #65731, #842, #29723, #58605, #22592, #59059, #87907, #23058, #51936, #80826, #44829, #73732, #23540, #52410, #3625, #47149, #52867, #75132, #74664, #61409, #17834, #45283, #23994, #38187, #82684, #4094, #54731, #89302, #81746, #24939, #53337, #82222, #9305, #76058, #53816, #90689, #39111, #10711, #74186, #10242, #90241, #46228, #68024, #11187, #31578, #46686, #75588, #3151, #31119, #24458, #39568, #67101, #25390, #68490, #32034, #16896, #2235, #45754, #17376, #60467, #60929, #88845, #89776, #9788, #32513, #54270, #25849, #40047, #83140, #68964, #38663, #18291, #67567, #32965, #61858, #2696, #16431, #60005, #85497, #69891, #76532, #5030, #41450, #19233, #63285, #20644, #49514, #63753, #76994, #34842, #92583, #19690, #27752, #78406, #29501, #70382, #5510, #83609, #48090, #85016, #91653, #13087, #41925, #33425, #13545, #34380, #70836, #11654, #92118, #42393, #47628, #26806, #71305, #35310, #77462, #27272, #40501, #49048, #5968, #56647, #12123, #6435, #40968, #84543, #69420, #55228, #33910, #77943, #4551, #84083, #64235, #93065, #18770, #62819, #55692, #48559, #62329, #56159, #12605, #91169, #26335, #20168, #37052, #8621, #38887, #24224, #80136, #51703, #59301, #51247, #2921, #45515, #73957, #88149, #74416, #67341, #15276, #1074, #45058, #37498, #8168, #10017, #80591, #73039, #59779, #44134, #87683, #15747, #88621, #23306, #22835, #53100, #81978, #23768, #52180, #74905, #58838, #44607, #66859, #65963, #81062, #73511, #52633, #1994, #29954, #30410, #38432, #30886, #66407, #81513, #1523, #67796, #16207, #16660, #9072, #31349, #37951, #9546, #17134, #2472, #87226, #58382, #60237, #89075, #46000, #22373, #15091, #15553, #23593, #24045, #80406, #51994, #30226, #8897, #88896, #74238, #44425, #60058, #59594, #43951, #31172, #9358, #66681, #423, #7517, #87498, #45337, #59117, #65316, #72399, #87958, #8442, #23111, #37775, #52920, #38242, #73331, #14646, #88444, #72848, #43503, #67156, #1808, #29310, #36402, #22647, #2289, #16029, #58204, #87048, #44880, #37321, #22197, #73782, #30694, #51066, #52460, #79953, #7976, #51519, #36870, #65785, #66229, #1343, #894, #81334, #16481, #29777, #58656, #83664, #17429, #82734, #9839, #53392, #32086, #47200, #45810, #82277, #47683, #69017, #69473, #46278, #75182, #60987, #4605, #39622, #10295, #11707, #40559, #26393, #60518, #89835, #62381, #76584, #38712, #39165, #17886, #74719, #81799, #4148, #3685, #46738, #33019, #90745, #67619, #24510, #68546, #24996, #31627, #33478, #68077, #2747, #83197, #89354, #3202, #53868, #18345, #75641, #10764, #91226, #16946, #76114, #32570, #61462, #90293, #25445, #54322, #11247, #40101, #61910, #25903, #54785, #18828, #27328, #36638, #65096, #55745, #29078, #91705, #73098, #63340, #79737, #43284, #29556, #41509, #5086, #15333, #57969, #84135, #66015, #7297, #62872, #86823, #19285, #84597, #56214, #65558, #1127, #85073, #196, #19747, #22429, #51301, #21981, #50381, #8228, #48615, #77515, #50855, #41020, #21504, #12665, #14879, #43733, #77046, #79285, #672, #72633, #70437, #7753, #26857, #37106, #92171, #58437, #72181, #87282, #5563, #33967, #44194, #80194, #48144, #55281, #36177, #34434, #12177, #69943, #14426, #30945, #38942, #39400, #2054 ),
 ( #68315, #30008, #59833, #88210, #44664, #58893, #81117, #88674, #23823, #2526, #16260, #52686, #67851, #74475, #67398, #80650, #17195, #60751, #66463, #81567, #23367, #74962, #31403, #87739, #37552, #51761, #60293, #17663, #22891, #9129, #1581, #38493, #66917, #16715, #15805, #89592, #89130, #10533, #45570, #24281, #73565, #9605, #10074, #53156, #82038, #24762, #45110, #46056, #2977, #31862, #8674, #38006, #53645, #30463, #82515, #46516, #75417, #59359, #52234, #74012, #4375, #18581, #47916, #10999, #4842, #61235, #3918, #33253, #12415, #12911, #69247, #40794, #19061, #91476, #77762, #63109, #62150, #70203, #19515, #18120, #55040, #91937, #55517, #82967, #90070, #76355, #34204, #76819, #54095, #25222, #11945, #90979, #27091, #69711, #84366, #46972, #33726, #55978, #75874, #11481, #84832, #48858, #26146, #83909, #39867, #62636, #48382, #26627, #90514, #5336, #32794, #77285, #68788, #61683, #47446, #41266, #25678, #54557, #19981, #41749, #3439, #83425, #40331, #32333, #87169, #28501, #42212, #553, #29435, #15219, #49338, #20925, #51189, #36522, #92404, #64046, #71602, #63579, #70662, #57849, #86235, #6736, #86703, #79627, #27564, #13371, #57393, #49794, #20471, #22318, #92887, #85321, #72072, #56460, #6256, #28048, #7189, #35609, #35124, #65438, #58326, #36064, #64525, #80076, #71126, #56938, #79164, #78232, #93350, #85775, #64981, #14310, #78691, #42683, #50743, #43171, #13832, #84, #21387, #5791, #50256, #28964, #21867, #43621, #14768, #72518, #34665, #7638, #72977, #53528, #9961, #2414, #29897, #36993, #23245, #74848, #88566, #1019, #8107, #23714, #37897, #38833, #59723, #31294, #65905, #52577, #67740, #58781, #52123, #2866, #89480, #66802, #30827, #87624, #9484, #60180, #67284, #37442, #45941, #73452, #45000, #22775, #15684, #88087, #38371, #51644, #44549, #31750, #89018, #60642, #8563, #66351, #81005, #24640, #1932, #1466, #82403, #44075, #80530, #30352, #16148, #59241, #73902, #9018, #81457, #16606, #45461, #74361, #24165, #53046, #81921, #17073, #26516, #10422, #53988, #4265, #90408, #61121, #62998, #39749, #32214, #18948, #3324, #46862, #68675, #47803, #47323, #75766, #77173, #12303, #76704, #11370, #34095, #18009, #10886, #26031, #89959, #18464, #3809, #11830, #54914, #39286, #83318, #91356, #83794, #32690, #40681, #82857, #91828, #25565, #69599, #33143, #84258, #61576, #25114, #70080, #4729, #46403, #26982, #62033, #54445, #33607, #75303, #76239, #40221, #55405, #55872, #69137, #62515, #90867, #19408, #17551, #41147, #48271, #5223, #68205, #5682, #42573, #64875, #93242, #85205, #57287, #27451, #7532, #92770, #14200, #71489, #57743, #71014, #34556, #43518, #86129, #19873, #437, #35500, #92294, #21278, #48743, #20355, #85669, #93701, #29325, #56828, #28395, #6620, #79049, #65333, #50634, #20817, #86588, #7083, #63465, #64415, #79524, #43061, #70558, #77647, #63932, #21759, #50150, #41639, #12798, #71965, #78582, #14663, #35956, #28857, #56343, #72416, #36417, #49227, #27938, #84724, #78124, #13720, #13262, #42099, #6146, #35017, #49687, #51081, #36884, #22211, #79969, #58218, #15106, #43966, #7991, #87062, #65799, #72865, #911, #41239, #18095, #82943, #3896, #70180, #11457, #25199, #77263, #12393, #91915, #32308, #32773, #34183, #19494, #75395, #46949, #54535, #46492, #53623, #40771, #69224, #83404, #69689, #62612, #10508, #90047, #40309, #61661, #3414, #5314, #75851, #68293, #55016, #39377, #10974, #39843, #83888, #18554, #68766, #48360, #63086, #19038, #47422, #82493, #54073, #90493, #62126, #61212, #76332, #25652, #47893, #90957, #4353, #33230, #26122, #84343, #17641, #33701, #76796, #4819, #91454, #11922, #26604, #55495, #65419, #78670, #42663, #27069, #85298, #28481, #35105, #50238, #79142, #70642, #55956, #14291, #84810, #5770, #71102, #48832, #77738, #19960, #64504, #41726, #6235, #20447, #50722, #12889, #42189, #34644, #43151, #86216, #63554, #71580, #63, #85756, #92383, #27542, #28027, #49315, #56435, #78209, #13348, #56916, #92864, #93330, #64024, #20904, #36045, #6716, #57374, #49775, #72054, #57830, #13811, #35590, #21368, #7170, #64962, #28944, #86681, #21846, #79607, #14748, #43603, #72499, #7617, #36503, #37422, #66333, #87149, #60160, #37878, #74829, #23224, #88547, #29415, #59221, #45440, #30331, #52103, #88999, #15660, #30805, #66784, #88067, #15197, #73433, #1914, #58306, #74341, #59703, #80988, #65887, #22299, #8086, #1446, #44529, #44982, #72957, #8543, #58761, #23695, #81437, #9942, #24146, #73882, #53024, #997, #16130, #29877, #16584, #45920, #87603, #38815, #52559, #2396, #80511, #51170, #9000, #9465, #22749, #38350, #67263, #80057, #31273, #81902, #17055, #51624, #44057, #36973, #531, #82835, #18446, #46382, #17988, #32194, #4245, #54897, #77155, #62497, #47304, #91336, #39266, #68652, #68183, #83774, #19390, #3304, #48253, #62014, #69582, #53968, #60622, #46840, #25546, #61099, #76219, #4710, #33588, #47785, #89938, #18930, #76686, #3787, #11811, #26498, #12286, #54427, #83298, #67719, #25094, #69119, #75743, #90849, #26011, #17532, #2850, #40662, #31731, #75282, #10866, #89460, #24621, #53506, #11349, #82382, #39729, #32671, #55389, #10401, #61557, #90390, #84240, #33125, #40203, #85652, #14185, #6130, #79509, #41130, #42082, #5664, #55856, #70063, #92279, #70998, #13246, #13704, #27435, #35001, #50132, #20800, #78566, #91813, #28378, #71949, #77629, #63917, #34540, #86113, #42556, #5204, #48727, #62980, #71473, #28843, #34078, #20339, #12779, #49670, #78105, #92754, #26965, #7069, #6605, #21743, #27922, #35483, #84709, #56810, #21262, #64399, #93225, #35940, #56327, #57269, #79031, #43046, #19856, #64858, #93685, #41621, #57727, #86574, #50619, #70542, #63448, #85191, #49209, #61594, #46422, #68223, #11389, #31770, #46882, #82875, #10440, #31313, #89499, #18028, #45480, #90427, #54008, #39306, #81940, #9507, #24187, #17573, #60662, #61142, #89037, #24664, #74870, #75784, #3827, #26051, #40241, #89978, #69156, #17097, #75323, #45963, #32708, #62053, #9980, #90888, #10904, #18482, #2885, #38395, #53550, #3343, #38851, #25132, #47345, #76261, #25583, #67759, #54466, #83336, #32234, #4284, #33162, #54938, #39772, #68696, #16626, #82423, #74379, #67305, #2433, #60199, #53065, #83817, #62539, #18970, #76725, #69621, #47823, #40701, #11851, #4749, #91380, #26537, #33629, #9136, #43290, #678, #36183, #8681, #44671, #72187, #30015, #52242, #44200, #23830, #79291, #80200, #43739, #202, #14433, #36644, #15339, #51308, #51768, #65565, #73106, #88218, #58899, #22897, #65102, #66471, #16267, #21987, #8234, #72639, #30470, #80658, #7303, #86829, #29085, #15813, #66924, #57976, #58443, #50861, #87745, #79743, #37112, #14885, #1588, #30952, #7759, #59840, #73572, #81124, #29562, #87289, #22435, #66021, #1133, #37559, #45117, #74019, #59366, #23374, #38013, #2062, #88681, #32801, #47454, #90986, #10541, #68322, #52693, #17202, #54102, #60758, #75881, #11006, #2533, #81574, #39875, #16722, #31411, #2984, #74482, #9613, #45577, #90077, #67405, #31869, #46063, #76362, #38500, #67859, #60300, #68795, #18127, #89137, #3446, #25683, #17670, #24288, #53163, #53652, #74968, #82045, #10081, #38949, #82522, #24770, #25229, #89599, #46523, #61690, #32341, #82974, #75424, #3925, #83432, #39407, #61242, #46980, #90521, #54564, #18588 ),
 ( #11488, #40338, #69254, #4382, #33260, #62157, #63586, #48866, #91483, #19068, #33734, #27098, #41274, #70669, #4849, #70211, #84373, #56469, #13377, #35617, #20932, #5798, #49801, #27571, #83916, #26634, #55985, #35131, #64532, #91944, #92411, #41757, #20478, #6744, #85782, #84839, #92896, #42219, #40801, #77770, #78698, #78239, #11952, #47923, #5344, #56945, #34671, #76826, #69718, #85328, #19988, #13839, #49345, #71133, #62645, #6262, #42690, #55524, #34211, #71610, #26155, #12918, #64054, #19522, #28055, #55048, #48389, #77292, #12422, #63116, #561, #21393, #64988, #43628, #58788, #57400, #91, #59248, #80537, #81012, #57856, #28971, #72525, #16156, #51196, #86711, #23253, #52131, #37904, #72080, #7645, #73909, #88094, #50263, #21876, #29445, #86242, #93357, #15692, #15226, #58333, #44556, #8570, #79172, #36071, #80083, #36529, #43178, #45007, #50749, #14318, #1026, #7196, #79633, #14775, #29904, #87176, #65445, #9025, #28508, #87632, #22325, #44082, #72984, #8115, #37001, #65913, #22782, #51651, #73459, #37449, #66358, #1473, #30359, #75310, #67292, #39293, #9492, #83325, #74856, #89967, #53536, #39757, #53053, #16613, #25572, #68212, #1939, #76247, #17558, #74368, #2421, #32697, #53995, #54452, #31301, #60187, #17081, #18471, #24648, #38379, #90415, #47331, #11378, #45468, #45949, #66809, #61583, #88573, #89025, #67747, #59731, #30835, #82864, #82411, #2873, #18016, #75773, #23721, #24172, #46410, #9968, #81928, #52584, #38840, #81464, #3331, #31757, #60649, #89487, #32221, #10429, #61129, #25121, #46869, #10893, #68683, #3816, #40688, #69606, #48751, #26038, #41154, #4736, #5690, #77656, #62040, #12310, #20365, #12806, #33615, #41648, #76711, #56837, #48278, #63473, #26990, #13270, #26524, #83802, #92778, #70565, #69144, #78590, #84731, #47810, #34564, #4272, #62523, #70088, #49236, #40229, #5230, #92302, #55879, #27459, #20825, #6154, #34103, #42107, #56351, #54922, #91835, #35026, #85213, #18956, #33150, #19415, #71022, #19880, #90874, #11837, #78132, #63005, #63940, #27946, #85677, #91364, #55412, #84265, #77180, #21766, #44446, #59138, #7539, #448, #71497, #72874, #918, #36891, #7092, #15576, #43068, #14670, #35508, #79057, #57751, #7998, #6629, #14208, #86596, #65806, #64424, #71973, #73352, #29797, #1365, #35963, #64882, #50641, #30248, #65341, #93708, #37344, #66250, #52017, #86137, #79531, #87982, #8464, #93250, #28863, #43525, #28403, #13730, #58677, #29332, #72423, #87523, #22668, #57295, #50159, #58225, #36424, #21286, #23134, #87070, #22218, #15114, #51088, #79976, #43973, #51541, #80430, #42582, #48045, #76950, #47582, #76007, #4979, #82635, #17785, #90643, #67974, #83093, #46638, #76486, #25805, #10193, #54225, #62280, #54685, #75539, #83559, #24889, #33865, #90196, #11609, #68918, #55181, #68440, #31984, #40925, #18719, #17328, #91608, #32920, #89725, #40454, #46178, #10663, #18248, #91115, #26763, #47100, #69372, #4050, #4502, #62775, #12077, #11138, #84040, #33381, #3101, #40001, #69846, #26285, #60877, #75083, #61362, #19185, #61810, #39062, #53769, #82171, #39519, #3573, #32463, #25344, #77416, #35264, #86372, #19647, #63713, #21523, #7318, #49474, #42352, #48516, #21060, #42827, #78824, #49004, #57527, #84970, #56603, #12555, #28181, #78365, #70340, #34798, #57070, #84501, #35743, #93024, #13504, #27228, #41405, #63243, #85457, #70793, #6393, #92074, #5928, #20119, #85908, #71743, #65115, #50401, #64192, #79307, #56117, #20604, #77902, #6871, #36196, #13045, #218, #49927, #14448, #41882, #5466, #92538, #71265, #27705, #13969, #43305, #72200, #64657, #93485, #28638, #55648, #58913, #9152, #23846, #67422, #80672, #44686, #29098, #87302, #30487, #37129, #52259, #81139, #72652, #57991, #16283, #86845, #7774, #73120, #50874, #79756, #22004, #66487, #43753, #8247, #22449, #52712, #14897, #44213, #36659, #45134, #88233, #65579, #73587, #2078, #87759, #694, #29578, #30031, #51321, #58458, #80214, #15353, #22913, #1149, #1603, #66036, #51783, #38031, #8696, #59382, #15828, #74035, #59857, #37576, #23391, #66939, #30968, #88698, #81593, #16742, #45598, #74498, #9630, #38517, #75441, #10098, #11025, #39424, #68341, #89156, #62175, #39894, #76844, #25247, #90542, #31429, #61260, #47473, #32360, #54123, #91007, #17689, #32818, #11971, #46998, #38965, #3946, #60318, #3000, #3466, #11507, #40819, #90096, #68815, #18144, #25700, #2550, #26175, #82994, #69272, #18608, #17218, #75901, #55066, #54582, #82061, #24305, #10559, #33280, #61708, #53183, #46079, #83454, #76380, #83935, #40355, #4401, #74987, #19088, #47941, #67877, #31886, #60777, #89617, #24787, #53669, #82538, #46539, #56961, #92912, #63135, #71627, #5363, #70687, #91498, #41293, #20010, #35151, #33752, #70228, #35634, #85798, #57420, #34229, #91964, #48888, #86259, #27593, #27119, #93375, #28525, #14335, #48407, #77789, #50285, #64551, #26654, #56003, #5817, #62664, #69738, #20949, #85348, #34691, #49817, #78714, #55543, #12445, #56489, #12937, #19541, #21410, #84858, #84392, #71151, #77310, #41777, #63605, #6280, #92429, #20496, #79191, #4870, #64072, #49363, #78257, #13395, #42238, #28074, #13856, #42711, #6760, #8584, #51664, #65005, #15240, #23267, #80553, #43645, #15708, #79648, #59743, #51210, #66371, #29918, #16169, #29461, #86728, #1957, #44569, #72096, #7213, #52596, #87647, #50764, #73472, #36086, #72541, #44096, #52145, #81477, #73002, #37462, #58802, #1489, #23733, #9038, #8130, #45021, #59263, #57874, #1040, #37916, #30372, #28986, #107, #22339, #73921, #22797, #21892, #14790, #88111, #37014, #66820, #81025, #30850, #7660, #88585, #43195, #36545, #80101, #65461, #577, #65928, #58349, #87190, #10179, #31969, #67959, #38117, #46622, #74118, #45684, #66565, #16365, #88781, #39048, #8779, #45216, #10644, #60862, #32444, #9238, #67027, #23929, #61345, #2633, #2163, #68425, #3555, #83077, #23475, #52799, #25328, #39504, #1687, #31053, #74591, #37657, #44768, #89705, #60400, #9719, #24872, #53754, #30568, #81219, #31512, #81678, #88319, #90180, #16827, #59466, #46164, #52341, #38599, #67503, #75067, #89238, #24391, #54208, #73668, #3084, #53269, #82152, #17307, #82620, #17767, #75522, #19167, #47561, #77395, #26742, #39982, #84019, #92052, #55628, #18698, #84477, #54666, #34776, #26263, #41383, #4959, #84947, #4483, #61790, #70773, #19627, #91092, #48979, #62753, #68897, #75987, #91585, #12057, #77876, #33844, #70316, #4029, #48496, #13024, #11115, #55157, #41860, #63691, #40904, #12532, #32902, #5446, #34314, #63220, #11588, #20097, #76466, #48024, #90622, #83539, #62259, #27206, #25785, #40435, #5906, #56093, #92516, #69353, #33360, #76929, #27682, #69824, #56580, #18230, #47081, #30001, #64167, #35718, #66008, #51294, #13483, #78799, #86346, #78341, #85433, #72626, #7291, #21497, #7747, #666, #42330, #28157, #72175, #64632, #35241, #37099, #13944, #6370, #86817, #71241, #21036, #42801, #21975, #50375, #49904, #80186, #15325, #50848, #79279, #8221, #85884, #71717, #190, #92999, #14420, #6844, #79731, #29071, #57047, #57502, #65552, #57963, #93459, #14873, #28613, #1120, #43277, #43727, #36170, #58430, #65090, #36631, #44186, #29550, #20582, #49453, #87276, #22422, #73091, #22884, #59351, #59826, #67844, #68308, #30937, #2519, #74467, #53149, #39393, #24756 ),
 ( #38935, #31396, #81560, #30456, #51753, #66456, #88667, #74005, #9598, #37545, #9122, #23360, #89123, #46050, #3431, #53638, #38485, #82508, #88202, #23816, #52227, #74955, #10526, #81110, #58886, #82030, #60744, #45103, #80643, #37999, #16708, #16253, #67390, #89585, #17656, #2970, #66909, #10066, #31855, #52679, #46508, #75410, #87732, #45563, #60286, #15798, #2047, #24274, #17188, #44657, #73558, #8667, #1574, #19508, #90063, #75867, #76347, #54088, #82959, #70655, #69704, #46965, #11473, #25670, #55971, #25215, #47438, #18113, #55510, #91468, #10991, #76812, #5329, #90972, #32326, #61228, #33246, #90508, #39860, #68782, #83418, #62142, #4368, #4834, #18573, #26138, #41257, #11937, #33718, #3911, #48376, #63101, #32788, #55033, #54550, #77278, #62629, #61676, #40324, #69239, #26619, #19973, #83902, #19053, #47909, #40786, #84358, #12407, #70196, #91929, #34197, #12903, #27084, #84824, #48849, #77754, #41742, #65431, #86696, #87162, #64037, #35117, #49787, #22311, #57387, #71118, #29428, #58318, #44068, #78224, #78684, #80069, #545, #27557, #92879, #6729, #92397, #5783, #21861, #21380, #35602, #50735, #14761, #56452, #42204, #86229, #13824, #49330, #51182, #28041, #20463, #7182, #85314, #56931, #85768, #36057, #64517, #20918, #15212, #34657, #64975, #93343, #63571, #6248, #42676, #14304, #13363, #28494, #71593, #78, #43164, #50250, #79156, #79619, #72065, #28956, #57842, #43615, #72511, #7631, #36516, #58774, #51637, #65898, #8099, #80523, #87616, #72970, #36986, #15676, #22767, #1010, #29890, #68880, #69336, #77378, #77858, #40418, #12041, #84003, #62737, #48961, #34297, #4467, #41366, #84460, #83060, #26247, #63204, #26724, #54190, #61326, #47545, #5431, #19151, #25312, #32427, #48007, #62241, #92034, #76911, #55611, #90164, #40888, #27189, #18214, #76449, #56076, #20081, #91076, #55140, #47064, #33828, #19610, #91568, #61773, #70300, #4010, #33344, #75970, #39964, #69806, #32886, #48479, #13008, #90606, #68409, #12516, #84929, #54649, #11099, #83523, #4942, #25767, #3538, #18681, #11570, #21958, #35224, #86800, #50831, #71700, #79715, #36612, #80169, #93442, #57486, #41844, #6351, #43261, #49887, #65074, #173, #85417, #70756, #29053, #5889, #20565, #85868, #63674, #92497, #34759, #79262, #56564, #21019, #64150, #65532, #27666, #57030, #49437, #57945, #7275, #78325, #86328, #14857, #6828, #13465, #42315, #42783, #92983, #71224, #28141, #78784, #35702, #13925, #14402, #64616, #28596, #43710, #21479, #72159, #50357, #72609, #7731, #36152, #649, #29532, #58412, #87258, #22404, #51276, #37082, #81541, #2950, #54886, #88181, #22865, #23797, #52209, #81091, #8203, #74936, #52661, #90840, #37980, #9577, #44166, #73986, #60266, #45085, #66888, #10046, #30438, #45544, #16689, #9103, #29983, #23341, #74445, #73072, #89103, #38466, #2027, #80623, #65991, #51730, #16235, #59330, #59808, #87714, #88649, #73539, #67370, #2499, #26001, #38916, #31377, #67825, #31836, #1102, #24255, #58867, #53129, #82009, #15779, #17166, #46031, #62005, #15307, #44637, #8648, #37525, #66435, #1555, #41121, #19847, #55847, #56318, #70053, #48718, #92745, #34533, #27428, #40653, #70991, #20793, #26489, #77621, #48245, #34994, #85183, #18921, #91327, #11802, #20332, #71465, #28370, #62970, #55379, #92272, #26956, #84700, #76677, #49664, #49202, #64392, #12770, #78098, #47775, #41612, #63910, #70534, #5658, #78559, #5195, #13239, #42075, #63441, #4701, #91804, #6123, #69572, #27916, #56803, #85645, #84231, #33578, #19381, #13697, #34068, #42549, #62487, #6597, #77147, #35475, #93218, #83765, #12277, #36860, #51984, #28834, #58194, #57718, #73323, #8889, #86564, #37767, #51510, #59108, #43494, #50124, #72390, #15082, #21733, #65776, #87950, #23102, #37313, #50610, #8434, #66221, #87038, #1335, #80873, #1800, #43942, #72839, #57262, #79500, #58646, #65305, #80398, #15543, #7061, #86105, #44415, #21254, #35931, #7507, #79022, #14176, #43038, #885, #71940, #36392, #14636, #30217, #412, #16021, #29299, #22188, #64849, #51056, #79944, #22638, #93676, #7966, #44872, #73774, #66672, #29768, #87488, #74711, #47192, #82268, #2281, #54314, #83189, #69009, #9349, #9832, #11238, #90285, #52452, #24036, #31620, #23585, #30685, #17878, #46270, #60511, #46730, #39613, #81326, #67147, #17421, #38705, #74230, #76105, #52912, #45329, #32078, #16473, #60050, #81791, #60978, #89346, #88888, #25436, #18337, #89826, #24502, #40093, #31164, #16939, #39157, #38234, #53383, #45801, #24987, #68069, #67612, #2740, #10756, #3194, #75174, #53860, #10287, #59585, #82726, #75633, #68537, #3676, #32562, #61454, #88436, #70428, #33011, #13587, #48606, #11699, #5554, #61902, #4597, #5077, #13132, #42439, #69935, #41499, #19738, #92162, #78451, #63798, #33959, #70881, #20215, #18818, #55736, #92627, #56205, #83654, #90737, #77038, #34887, #77506, #54777, #25895, #12653, #91696, #27798, #34424, #85064, #47675, #63331, #56691, #76576, #12169, #85538, #49556, #26848, #84588, #40550, #27319, #49093, #69465, #33470, #20686, #77992, #4140, #62373, #91216, #48135, #26384, #41968, #55272, #84127, #19277, #41012, #62863, #6012, #51868, #37209, #93108, #64735, #72276, #64279, #15912, #58539, #86929, #7395, #87384, #80295, #28263, #14052, #58076, #50487, #21142, #22993, #93563, #85992, #72733, #57152, #6948, #28720, #7853, #36277, #35821, #1230, #30112, #36740, #65197, #87843, #71829, #57605, #79835, #50012, #300, #86448, #65661, #14975, #78905, #43381, #51403, #43831, #21606, #775, #42915, #80760, #79389, #29659, #22082, #44300, #14526, #29180, #58994, #22531, #6480, #71349, #50952, #15434, #73208, #35357, #8327, #14995, #23011, #23494, #79856, #51423, #29678, #8346, #88343, #73687, #43854, #80783, #30131, #28743, #65684, #8797, #66134, #93584, #6969, #86950, #44786, #58561, #64759, #71849, #87402, #7873, #37676, #22549, #1249, #35842, #15452, #66585, #57626, #22103, #1705, #59490, #36763, #798, #86469, #73235, #59015, #37229, #7417, #15932, #43402, #72752, #21634, #79411, #58104, #87862, #320, #44323, #51890, #30588, #29204, #52362, #14077, #42942, #50513, #14546, #72297, #36299, #50972, #31530, #52817, #60879, #10195, #81237, #59959, #9257, #39064, #68442, #16384, #67521, #88798, #75085, #2651, #60417, #38134, #10666, #67977, #61364, #24408, #31986, #74139, #53287, #53771, #89257, #82173, #39521, #9742, #3103, #89727, #17330, #2186, #38617, #24891, #45234, #75541, #82637, #17787, #45701, #31071, #16845, #46180, #46640, #3575, #81697, #32465, #67049, #23945, #74613, #26056, #85698, #70583, #20844, #91386, #27008, #55429, #13289, #42603, #84282, #71518, #85235, #56857, #12327, #83823, #41171, #48768, #48296, #5709, #49715, #13755, #71043, #70110, #6177, #63960, #19897, #54943, #18975, #47828, #77674, #34584, #76730, #5250, #27479, #63022, #49256, #78151, #40706, #11857, #69626, #4754, #71995, #14691, #7113, #43546, #8940, #58699, #36446, #65361, #87092, #88005, #57316, #22242, #15136, #51563, #30269, #23158, #16071, #44925, #73827, #64445, #93271, #38758, #2337, #52501, #66725, #25037, #61031, #31216, #39668, #67201, #67662, #59642, #9404, #81842, #3244, #1852, #38288, #3726, #53909, #25487, #60101, #88940, #16992, #54366, #89400, #24088, #61501, #90333, #76156, #16526, #45857, #18387, #32611, #88489, #52965 ),
 ( #32135, #31669, #83240, #74763, #9882, #46322, #23636, #2788, #60562, #89877, #75226, #81378, #24554, #17929, #10340, #53438, #39206, #74281, #47244, #82321, #82776, #17472, #10806, #68119, #45378, #37818, #46780, #30739, #75681, #68590, #18869, #12709, #69059, #11749, #12218, #20266, #20732, #77087, #48659, #26898, #5601, #85585, #70930, #41064, #78039, #27367, #25948, #62911, #6061, #63381, #90788, #4188, #84176, #42014, #55786, #61951, #33062, #84639, #5130, #34933, #19788, #92211, #54829, #77560, #63848, #83707, #19324, #92680, #56739, #34007, #91747, #47726, #70473, #26433, #41549, #34475, #56256, #76626, #48186, #85116, #40143, #49142, #13179, #27850, #40602, #69516, #4647, #69990, #55326, #49602, #33522, #11289, #62428, #91269, #65712, #87886, #73261, #58129, #8373, #50060, #79437, #78956, #824, #30156, #14106, #59039, #72777, #80338, #64786, #71400, #93611, #36327, #42970, #86974, #15480, #44351, #58588, #71875, #29705, #87427, #14573, #22574, #37253, #23039, #65241, #347, #78498, #6997, #79881, #86500, #7902, #36792, #28310, #13636, #51448, #42487, #57199, #28769, #6533, #35409, #64329, #22128, #93155, #57652, #35869, #66158, #86040, #21663, #21189, #1274, #43881, #50539, #29234, #43429, #72324, #7445, #50996, #15021, #16410, #66608, #80807, #9282, #81724, #23973, #24434, #38165, #16873, #60908, #2676, #89282, #8823, #39088, #82661, #88369, #45731, #45262, #3130, #53316, #15956, #59520, #73713, #82200, #39546, #90220, #31098, #23519, #60447, #88824, #52847, #44811, #17810, #17355, #32491, #74642, #46206, #37703, #9768, #32010, #38644, #67547, #46663, #75567, #51917, #30618, #2214, #61388, #10689, #1731, #74166, #31555, #52388, #81265, #68001, #75111, #10221, #89755, #24916, #67080, #59985, #53793, #68469, #3604, #70817, #47608, #40027, #26786, #11167, #54709, #76511, #55673, #55207, #83586, #84992, #20147, #84524, #19210, #41904, #25830, #18750, #33890, #68944, #26312, #11634, #19671, #62797, #47125, #91145, #5488, #91632, #40480, #48539, #61837, #5950, #33406, #77440, #12102, #92097, #69397, #4074, #77926, #12584, #54250, #34822, #69869, #32945, #41431, #83120, #4529, #84061, #34361, #63735, #48069, #70363, #40947, #63266, #25369, #49030, #76972, #27253, #56139, #90670, #5007, #13068, #18271, #62305, #76038, #71767, #29599, #43325, #49496, #56628, #72221, #86392, #58478, #14468, #50894, #20625, #7337, #87322, #85478, #6890, #22470, #44234, #21543, #79331, #78385, #58014, #79775, #22024, #85930, #714, #28202, #93504, #13526, #64215, #42851, #86870, #42374, #93045, #51342, #14918, #80236, #57090, #21080, #35764, #15372, #50426, #49951, #73143, #78844, #64677, #8269, #36217, #13990, #37149, #92560, #27731, #71286, #28659, #6413, #35288, #57547, #65137, #238, #29118, #43773, #72674, #7794, #36679, #65601, #75007, #58933, #8718, #52733, #45157, #15849, #17708, #88257, #80695, #67443, #51803, #1625, #23415, #2570, #2101, #30508, #31907, #60799, #31449, #59879, #82560, #66506, #59403, #74520, #44706, #66962, #52281, #60338, #9655, #87783, #38053, #46102, #38540, #81160, #89175, #37595, #46561, #74056, #24327, #81616, #38985, #16304, #73607, #24807, #53204, #1169, #75460, #16765, #9175, #82082, #30052, #30992, #88719, #10119, #10581, #23867, #17240, #45618, #67898, #66056, #89637, #3021, #53693, #22933, #54145, #91027, #5386, #91521, #25268, #32381, #18631, #70251, #83959, #90116, #3488, #19108, #33299, #34251, #55090, #26677, #61282, #47963, #63157, #83014, #47497, #91988, #84881, #62197, #26196, #18166, #4891, #55567, #62688, #32840, #41314, #68838, #40375, #47019, #11047, #83475, #33775, #75921, #39917, #27141, #84415, #56026, #3966, #20032, #48909, #61730, #90562, #69292, #25720, #77811, #19563, #76867, #4421, #48429, #77333, #54604, #76406, #11992, #11528, #40841, #39444, #69760, #12467, #68360, #92452, #42264, #64096, #14357, #42733, #71177, #72563, #7685, #72118, #6781, #29485, #13419, #6306, #21435, #27615, #13880, #35174, #7234, #50309, #34713, #78737, #86751, #79214, #92936, #43217, #49389, #58370, #20973, #36109, #93398, #79672, #28097, #56512, #65485, #65027, #41799, #22360, #57441, #20521, #127, #70710, #56984, #71648, #21913, #51234, #35658, #29010, #28550, #57895, #87212, #36570, #64573, #14813, #50787, #85371, #86282, #602, #43668, #78281, #5841, #85822, #12960, #63627, #49840, #45393, #32147, #75238, #18398, #3257, #39680, #9417, #61046, #47257, #74293, #89412, #76170, #33075, #10353, #68136, #38303, #46793, #68603, #10820, #74778, #83254, #17004, #82334, #67218, #52980, #31683, #75695, #2351, #81854, #11302, #3739, #69072, #45872, #9896, #60577, #4200, #39218, #38770, #40155, #61964, #25960, #60114, #24566, #31228, #90801, #67674, #88953, #82790, #24100, #2800, #53453, #17942, #17484, #46336, #80122, #15261, #32623, #89890, #25049, #53922, #61513, #90345, #25500, #54378, #84189, #20286, #63398, #76636, #26913, #34951, #92227, #55338, #27383, #91282, #71416, #62927, #78054, #41566, #27866, #41079, #4662, #13652, #56273, #83722, #64348, #5617, #62440, #85132, #18882, #19337, #55800, #63863, #93175, #84652, #49160, #70489, #13195, #35426, #20748, #19804, #56759, #70945, #69529, #12723, #49619, #42031, #40613, #47738, #34022, #85601, #34492, #11761, #33535, #6077, #48672, #78515, #92697, #42504, #26448, #6548, #54841, #48200, #91761, #77101, #12232, #77573, #70003, #5145, #87445, #15496, #51466, #21680, #30173, #57672, #29250, #50077, #93628, #72342, #22591, #86057, #28786, #87904, #44367, #15974, #86516, #50556, #7461, #44827, #79899, #79453, #51934, #80824, #66626, #7015, #36343, #8842, #23056, #78972, #14589, #58145, #21207, #28327, #73278, #43897, #86991, #8390, #37269, #14124, #64804, #15037, #65258, #42988, #57217, #66175, #72794, #22144, #1291, #59056, #71894, #43446, #7918, #364, #35887, #73730, #51012, #36809, #29722, #65729, #840, #58604, #80355, #37720, #60003, #61406, #90239, #60927, #89300, #18289, #2233, #31116, #10240, #81283, #2694, #88843, #89774, #39108, #23537, #67565, #75586, #68022, #23992, #3149, #38184, #47146, #9786, #24937, #82220, #68487, #81743, #45281, #54268, #32031, #30638, #11185, #46226, #9302, #53814, #59537, #52865, #31576, #10709, #40045, #60465, #82682, #17374, #17832, #76055, #25388, #24455, #3623, #46684, #16429, #53334, #83138, #39565, #74184, #88387, #74662, #32510, #75130, #52407, #67099, #1750, #16893, #45750, #38661, #27269, #90687, #48556, #5965, #32963, #76991, #34839, #20641, #62816, #55689, #61856, #34377, #56156, #92115, #62325, #70833, #4548, #69887, #25847, #40499, #19229, #63282, #54728, #69417, #63750, #85012, #56644, #33422, #91165, #48087, #85494, #26803, #26332, #92579, #27748, #13542, #47626, #12120, #49511, #78403, #83606, #55225, #5026, #84079, #68961, #4092, #20164, #91649, #18768, #40965, #33907, #77457, #76529, #84540, #19687, #49045, #12601, #11652, #41447, #77940, #70379, #5506, #13084, #41922, #58950, #50443, #65616, #29135, #15386, #28675, #85945, #1184, #14933, #71302, #51821, #86884, #49966, #43788, #6431, #42867, #43339, #51359, #80713, #14481, #79791, #58030, #36696, #22947, #8283, #72236, #44251, #58492, #57106, #253, #37163, #728, #28218, #35306, #21559, #73163, #22038, #93062, #64232, #50907, #36232, #66072, #72688, #29614, #21098, #7807, #30065, #78857 ),
 ( #87798, #87337, #14007, #42390, #71781, #6903, #35778, #86405, #64691, #93517, #57562, #79346, #7350, #65150, #22486, #80250, #31466, #45633, #3038, #24824, #8735, #52298, #2586, #88736, #59422, #61298, #38070, #30522, #17259, #1642, #45171, #66980, #46118, #74541, #90133, #2118, #88274, #75021, #23430, #74073, #31008, #10134, #9672, #9192, #75476, #10601, #39000, #38555, #32399, #16319, #59894, #24344, #81175, #16779, #23882, #67914, #53219, #37612, #81632, #89655, #82100, #52750, #31921, #67457, #25284, #60354, #60813, #89191, #82575, #53708, #17723, #68377, #46578, #44723, #54161, #39460, #3507, #15866, #73623, #66523, #83975, #92004, #92466, #55109, #26694, #4907, #77349, #63644, #48928, #19123, #56045, #5402, #3981, #40859, #77826, #41333, #68852, #75937, #62212, #20048, #33792, #39935, #47036, #62707, #76882, #12976, #91537, #70268, #11065, #55583, #41814, #32856, #91042, #70725, #34728, #12009, #69777, #61745, #48448, #34267, #12483, #76421, #84899, #18648, #47978, #90577, #54619, #33316, #63174, #25737, #83491, #5857, #27157, #27632, #47515, #11543, #26214, #83030, #84431, #40390, #18184, #69308, #4436, #19579, #6799, #37053, #22375, #78296, #49855, #57456, #49406, #1075, #43681, #72131, #86298, #72577, #65498, #13435, #92952, #43233, #35673, #6321, #42282, #28565, #36584, #65040, #57000, #29023, #28112, #73040, #64588, #79685, #7247, #29502, #42749, #35189, #15277, #57910, #85387, #65964, #36123, #64115, #86765, #20536, #85837, #21451, #616, #56530, #50324, #143, #21927, #50800, #71194, #51248, #79230, #58383, #7699, #20988, #14372, #80137, #14827, #78754, #13895, #93413, #87227, #44135, #71665, #8169, #74418, #23769, #60700, #45516, #81979, #51704, #9547, #89539, #87684, #37953, #24703, #75362, #52634, #16661, #22836, #89076, #17136, #53101, #23307, #31807, #59302, #30887, #80592, #1525, #73958, #24225, #15748, #30411, #53588, #46001, #17609, #88150, #52181, #9073, #46460, #81514, #81063, #82461, #10477, #68262, #8622, #66860, #39343, #29955, #44608, #16208, #59780, #73512, #58840, #74906, #38433, #88622, #10018, #38888, #37499, #66408, #67342, #1995, #45059, #2473, #31350, #60238, #67797, #2922, #68734, #61633, #19009, #76302, #3865, #84313, #19464, #47862, #40279, #41209, #39812, #32745, #26092, #54043, #11427, #90466, #76765, #54981, #47391, #90015, #10946, #54505, #11893, #32272, #25623, #48331, #40742, #77232, #83376, #18525, #69196, #70147, #4325, #33202, #12361, #5283, #34152, #46920, #62093, #3384, #61178, #75822, #90926, #83857, #82913, #25169, #55463, #69659, #4789, #18067, #33669, #26574, #62579, #91421, #67185, #37803, #39651, #16512, #8925, #89383, #73812, #23620, #45363, #24538, #24073, #52487, #53894, #82762, #53422, #81826, #10790, #88473, #81362, #2773, #66709, #88925, #74266, #82305, #31654, #16056, #60086, #68104, #60545, #9389, #17456, #30725, #68574, #2320, #46306, #74746, #61016, #38273, #1838, #46765, #75210, #23143, #3711, #38742, #59625, #10325, #52025, #31201, #52949, #3229, #32596, #16977, #39192, #9867, #32120, #87990, #17914, #45842, #89862, #25022, #67647, #75666, #80911, #44909, #47230, #54351, #40587, #92196, #12203, #18370, #25472, #41047, #55308, #27352, #77072, #19772, #83225, #69974, #56239, #76140, #69501, #85101, #13163, #84161, #48171, #11274, #26884, #48642, #84624, #54814, #63366, #90772, #91254, #19309, #20251, #76611, #91731, #33992, #5114, #40127, #4632, #62895, #90318, #41533, #55771, #77543, #33046, #69044, #4173, #62412, #11734, #12693, #61936, #33506, #25931, #70459, #5586, #70913, #49127, #34458, #78023, #83692, #26418, #18853, #41999, #6046, #47711, #61486, #29216, #36775, #21174, #27835, #50043, #86481, #64314, #14557, #65695, #809, #15007, #28294, #79867, #43866, #64771, #72763, #29689, #73246, #21646, #50524, #34918, #93139, #36310, #42954, #58115, #86960, #78483, #63831, #22113, #92663, #13619, #78939, #56724, #85570, #20717, #72309, #49587, #14089, #57184, #58573, #42472, #71860, #71383, #50982, #331, #6516, #79422, #7885, #93596, #35394, #86025, #35854, #6981, #28754, #57637, #43414, #7430, #65226, #87413, #22560, #51434, #80323, #15463, #44335, #59026, #89268, #39074, #44796, #67062, #66595, #53299, #9754, #37240, #15942, #30142, #74625, #89739, #46650, #81248, #73699, #16857, #45246, #74151, #1260, #67987, #45713, #82648, #31082, #2661, #66144, #2198, #82184, #81708, #3113, #31996, #17340, #1716, #46191, #75096, #38146, #10205, #60889, #8357, #59970, #23955, #87873, #30600, #38628, #16395, #31540, #60428, #51901, #23023, #24418, #80794, #8808, #52373, #37689, #59503, #88354, #67531, #23505, #9268, #88808, #24901, #52830, #53781, #17797, #6284, #42242, #39531, #27595, #49821, #41779, #21414, #75552, #77791, #41295, #90207, #10676, #34231, #12940, #48890, #49367, #63137, #70689, #85802, #56492, #20499, #32477, #64076, #13859, #19543, #5819, #70230, #28077, #78261, #68453, #83105, #3587, #13398, #64555, #61374, #56005, #48409, #85351, #20012, #34693, #25356, #42714, #71155, #57423, #63607, #35155, #54236, #92431, #56965, #92915, #20953, #71631, #91966, #78718, #6763, #35637, #77312, #84861, #93379, #12447, #28530, #86263, #5365, #27122, #43198, #57877, #51213, #65465, #1043, #28989, #582, #14794, #80558, #37466, #59747, #45024, #29922, #73924, #21895, #80104, #50768, #66375, #1961, #79653, #30854, #44573, #52148, #36549, #72099, #29465, #8134, #43649, #50289, #1492, #14339, #110, #58354, #7216, #36089, #88588, #87650, #65009, #87194, #72545, #9041, #86732, #22342, #7666, #73476, #15712, #15243, #58806, #23272, #44100, #79196, #73006, #37017, #65931, #22801, #51668, #8588, #30376, #59267, #88115, #81028, #16172, #37919, #66823, #61146, #74382, #10908, #54471, #60202, #82426, #81943, #68702, #25135, #52599, #31316, #45483, #89981, #11394, #62058, #2888, #89040, #32237, #60665, #89502, #16629, #83341, #54011, #4289, #46425, #18032, #81480, #17576, #3832, #53554, #75327, #18487, #38855, #82878, #46886, #10443, #38399, #31773, #75788, #9510, #32714, #39776, #39309, #24190, #67308, #53068, #24667, #67762, #68226, #2437, #3346, #17100, #61599, #90432, #33167, #47350, #25588, #76267, #45967, #40246, #74873, #69162, #23736, #9983, #30498, #73130, #80682, #65124, #71755, #227, #36669, #14457, #58467, #15838, #44695, #58922, #72210, #30041, #87770, #14907, #22922, #73596, #23403, #65590, #704, #78833, #43314, #80224, #86858, #8257, #37138, #28647, #36206, #43763, #51792, #29588, #22458, #35753, #66046, #8707, #21532, #72663, #7326, #37585, #15361, #13979, #86381, #6880, #51331, #66496, #42838, #58002, #50413, #87311, #22013, #50883, #64666, #1613, #44222, #59392, #7783, #1158, #93494, #88244, #57537, #79319, #29107, #79765, #67432, #82547, #24794, #46089, #66950, #31438, #53679, #81149, #32368, #89626, #74996, #23856, #45146, #59868, #53193, #2559, #3010, #30979, #60328, #16753, #17697, #39433, #61717, #47007, #31895, #75911, #52722, #82071, #81605, #68349, #3955, #45608, #32828, #46549, #54132, #38528, #74045, #89165, #10108, #74510, #60788, #83002, #18154, #61269, #9641, #3477, #90104, #17227, #25255, #11036, #90550, #38975, #67887, #52269, #24315, #75450, #10568, #39904, #68825, #2089, #16293, #9163, #38042, #88708, #69746, #47483, #76392, #64082, #63144, #40363, #4878, #19097 ),
 ( #5827, #47950, #70696, #34699, #55552, #63613, #20505, #25709, #77319, #41301, #54591, #83944, #27128, #33762, #48896, #77797, #69280, #83463, #12947, #18619, #4409, #62673, #11516, #33288, #62183, #91974, #91016, #91507, #76853, #49374, #26184, #40827, #55075, #41785, #84867, #11979, #70237, #92437, #84401, #26663, #19550, #48416, #12453, #5371, #34238, #56011, #20018, #27601, #56498, #85357, #78267, #13406, #42249, #71162, #6290, #35160, #31217, #36915, #59161, #58700, #45379, #1853, #28082, #8020, #22243, #66726, #81843, #38759, #73374, #65832, #8941, #37365, #66272, #87093, #60102, #37819, #74765, #23159, #88490, #58249, #88006, #74282, #30270, #52043, #88941, #15596, #30740, #59644, #80928, #15137, #8486, #23637, #51113, #9405, #52502, #16072, #939, #79999, #29818, #1387, #44469, #44926, #72896, #73828, #87543, #81379, #16527, #9883, #24089, #38289, #52966, #22690, #67203, #51564, #2338, #45858, #80451, #92921, #16993, #43999, #53910, #60563, #46781, #4648, #18388, #24555, #31670, #47245, #61502, #33523, #83241, #25949, #89401, #76157, #62429, #53439, #75682, #91270, #19325, #90334, #54367, #82322, #33064, #54830, #90789, #61032, #69517, #3245, #68591, #17473, #39207, #17930, #61952, #46323, #68120, #26435, #83708, #55327, #32136, #89878, #10807, #84177, #25488, #25038, #48187, #77088, #12219, #75227, #39669, #67663, #2789, #10341, #82777, #3727, #32612, #11290, #18870, #40144, #69060, #47727, #76627, #4189, #11750, #40603, #20268, #84640, #86502, #63383, #55787, #42489, #26899, #70475, #92213, #71402, #70932, #5603, #6999, #35871, #6535, #34935, #57654, #41551, #34477, #49604, #19790, #42016, #27369, #35411, #78500, #62912, #13182, #21191, #13638, #56258, #64331, #77561, #21665, #49144, #93157, #27852, #14108, #85118, #48660, #93613, #28312, #69991, #50541, #85587, #12710, #57201, #5131, #78041, #6063, #50062, #79439, #63850, #86042, #56741, #78958, #41065, #64788, #92682, #42972, #71877, #20734, #28771, #34008, #91748, #349, #7447, #30158, #8825, #88826, #74168, #44353, #81267, #30620, #29236, #66160, #9284, #66610, #58131, #36329, #87429, #45264, #59041, #65243, #72326, #87888, #8375, #38167, #23041, #1733, #86976, #51919, #67082, #22130, #22576, #2216, #59987, #37255, #1276, #50998, #73715, #59522, #37705, #7904, #16412, #43883, #15482, #79883, #15023, #58590, #88371, #72779, #36794, #31100, #23521, #23975, #65714, #826, #51450, #52849, #80809, #29707, #14575, #43431, #80340, #73263, #15958, #44813, #52390, #9770, #75113, #82663, #74644, #26314, #68946, #3606, #17812, #4076, #90672, #38646, #24436, #68471, #60910, #31557, #33408, #10223, #2678, #83122, #67549, #17357, #39090, #18273, #46665, #46208, #47610, #76513, #47127, #75569, #4531, #82202, #68003, #90222, #60449, #10691, #3132, #76040, #25371, #89284, #53795, #61839, #54252, #32012, #11169, #53318, #62307, #89757, #40029, #32493, #54711, #24918, #39548, #40482, #32947, #16875, #91147, #61390, #25832, #83588, #45733, #18752, #11636, #69399, #81726, #27255, #92562, #78387, #20627, #19212, #5951, #28204, #20148, #93505, #55209, #56141, #19672, #69871, #84063, #12586, #84994, #49031, #27732, #41433, #77927, #64217, #34823, #56629, #12104, #42376, #85932, #91634, #13070, #48541, #6415, #85480, #48071, #62799, #76974, #13527, #42853, #40949, #34363, #26788, #63736, #92099, #41906, #5009, #21082, #71288, #35765, #70819, #35290, #33892, #93047, #57092, #49953, #78845, #13991, #70365, #71769, #6891, #64679, #55674, #63268, #84525, #77441, #5490, #66058, #51344, #239, #21545, #36218, #29601, #43774, #73145, #7338, #72676, #86871, #58934, #15850, #38055, #23417, #8271, #52282, #29120, #58480, #58016, #44708, #74057, #22026, #9177, #22935, #30509, #14920, #50428, #7795, #80237, #50895, #37151, #59405, #88258, #8719, #79778, #73609, #37597, #87324, #66507, #81162, #66964, #15374, #44236, #28661, #36680, #30053, #65602, #51805, #80697, #72223, #57548, #1627, #86393, #65138, #716, #79333, #14469, #43326, #1171, #22472, #87785, #16306, #45158, #59881, #17242, #52735, #23869, #75462, #32842, #88721, #10121, #61732, #47499, #89639, #82562, #81617, #61284, #83016, #25270, #89177, #3968, #31451, #3023, #16766, #67445, #46104, #90118, #45620, #2572, #90564, #18168, #83477, #60340, #24329, #75009, #18633, #53695, #53206, #25722, #54606, #40377, #74522, #38987, #76408, #11530, #9656, #82084, #31909, #38542, #2102, #47021, #17710, #60801, #75923, #11049, #67900, #24809, #46563, #10583, #39446, #30994, #68362, #3490, #32383, #54147, #39919, #68840, #70713, #5389, #33778, #35177, #64099, #34716, #63160, #85825, #69763, #4894, #77814, #55092, #70254, #62691, #63630, #12963, #91029, #41317, #49392, #41802, #91524, #5844, #11995, #20976, #77336, #92455, #56029, #42267, #55570, #19110, #28100, #27618, #4423, #13883, #20035, #76869, #56515, #33301, #26680, #34254, #78284, #69294, #91991, #85374, #84884, #20524, #49843, #92939, #27144, #71180, #13422, #83961, #48912, #56987, #6309, #47965, #62199, #48432, #26198, #40844, #84418, #19566, #12470, #93401, #21438, #28553, #86285, #57444, #35661, #50312, #79217, #42736, #71651, #6784, #64576, #68931, #74628, #3115, #2663, #83107, #39533, #67065, #45715, #59972, #10678, #25817, #76497, #17342, #9756, #46652, #75098, #10207, #31084, #4062, #75554, #18734, #60891, #32479, #2200, #31998, #18259, #67989, #89742, #32932, #53301, #68455, #3590, #24903, #52832, #46193, #61376, #88810, #47112, #90209, #53783, #38630, #23957, #67533, #39076, #82187, #82650, #16859, #17799, #31542, #25358, #54238, #47595, #61824, #76020, #90656, #60430, #11153, #89270, #40014, #83572, #24420, #38148, #54697, #81710, #91619, #4516, #26774, #63254, #40937, #84981, #42362, #71275, #85467, #4992, #56616, #20614, #41419, #49484, #6402, #49938, #92085, #27240, #11621, #69857, #13057, #19658, #34811, #63724, #55193, #40466, #92549, #69384, #19197, #55659, #33393, #62292, #91129, #49018, #26300, #84512, #33878, #35275, #48057, #48527, #76961, #27717, #70804, #12089, #56128, #78374, #70351, #62786, #77428, #12569, #5477, #34347, #20133, #77915, #41893, #5939, #85918, #64204, #13513, #93034, #28190, #57079, #21069, #35203, #63656, #77840, #64132, #57013, #40871, #84443, #92479, #27170, #91550, #93426, #70281, #62720, #49418, #33807, #77361, #5414, #78308, #12988, #12495, #13908, #42761, #13447, #41826, #64601, #48461, #41348, #56545, #26707, #48941, #34279, #42297, #85400, #69789, #20059, #28124, #20548, #63187, #71207, #19592, #28578, #56058, #6334, #27644, #21002, #92017, #55595, #6812, #92966, #76894, #57469, #85849, #84912, #49868, #12023, #70737, #5871, #78767, #86311, #71681, #35686, #47990, #4920, #2007, #81075, #51260, #88162, #37510, #36136, #73053, #16219, #73524, #7259, #14386, #631, #52193, #65975, #72143, #79244, #1086, #15291, #45070, #37066, #8633, #43245, #29967, #73970, #65054, #29516, #9086, #66871, #44148, #8184, #156, #80604, #66420, #44622, #14840, #23322, #50814, #22388, #29036, #86782, #65511, #15762, #57924, #21941, #37964, #1538, #30901, #79698, #43693, #58396, #59792, #58852, #72591, #21463, #50337, #7712, #36596, #87242, #80152, #87697, #22849, #51715, #30422, #59313, #33212, #75833, #10487, #24715, #10956, #3877, #81525, #31361, #75374, #67808, #38447, #40290, #17147, #9559 ),
 ( #61190, #60250, #11439, #2933, #18077, #39355, #61643, #74918, #67354, #47402, #90027, #23781, #4335, #68272, #2484, #25179, #52645, #89087, #89549, #32755, #88633, #60710, #32283, #3394, #82923, #69206, #54516, #53600, #90476, #39823, #24237, #46470, #83386, #46930, #74429, #16673, #31818, #25633, #54053, #45528, #53113, #68747, #82472, #18536, #76313, #81993, #46014, #10029, #38899, #17619, #70159, #92846, #13796, #55938, #48815, #26103, #27527, #49299, #85280, #55476, #64008, #91434, #63067, #83868, #33682, #12374, #56420, #54995, #62590, #28010, #78194, #49761, #26586, #84325, #41221, #78656, #19943, #19475, #85742, #20888, #6700, #40753, #5295, #19020, #12871, #84793, #56902, #77720, #20430, #47874, #41710, #42648, #76777, #34165, #71565, #62107, #70627, #5753, #11904, #13332, #42174, #71087, #48342, #90939, #77243, #91896, #69670, #27051, #34628, #6220, #4802, #63539, #92365, #35089, #23210, #49, #64948, #79594, #52090, #87135, #7156, #59207, #88053, #73868, #14275, #14735, #16117, #1433, #57361, #28929, #36489, #28467, #35574, #22735, #51157, #65406, #51608, #44514, #86203, #72040, #22286, #43589, #79128, #80973, #57816, #50224, #36959, #21353, #86667, #21831, #65872, #517, #50706, #30317, #44968, #981, #29400, #64490, #36030, #72486, #44043, #43135, #58292, #7602, #29862, #72945, #80044, #15184, #15645, #8070, #58746, #87589, #80497, #93316, #73419, #8529, #37408, #66317, #88985, #52546, #61543, #75270, #37865, #18429, #53492, #16571, #10386, #66769, #9451, #9928, #17972, #47287, #74813, #46368, #24604, #3287, #83284, #68638, #38802, #75727, #25079, #23681, #60608, #3770, #61081, #88533, #1901, #81886, #39714, #82368, #59690, #67706, #46825, #17518, #39252, #81421, #89923, #32655, #45426, #2834, #67250, #53953, #68167, #30791, #74326, #38337, #32180, #90376, #8986, #17041, #2381, #82820, #45907, #31717, #31260, #25531, #10849, #60147, #89444, #54412, #24133, #53011, #27417, #12268, #34058, #70979, #91319, #12760, #48705, #70042, #90833, #55370, #77609, #11334, #56305, #19837, #5184, #47769, #69105, #83758, #77137, #26480, #26945, #54879, #84222, #40645, #41601, #63431, #85635, #6112, #55833, #34983, #76668, #41110, #11795, #92260, #27905, #69565, #56793, #70523, #78087, #62478, #4231, #19369, #62960, #4693, #84688, #13230, #42065, #85171, #33568, #20322, #49192, #91794, #63897, #92733, #20782, #5649, #34524, #76205, #48234, #40186, #33109, #61998, #25993, #18914, #49654, #36848, #13686, #93208, #93664, #71449, #6586, #87937, #87026, #64383, #28824, #43027, #73311, #42538, #64839, #35464, #72828, #15069, #28360, #398, #22624, #14625, #78548, #57252, #50596, #14163, #86094, #21244, #7052, #79490, #21721, #22177, #35921, #50113, #71930, #51045, #57707, #7953, #65765, #79008, #86550, #875, #43483, #72379, #7496, #36381, #65294, #29288, #79933, #58184, #43931, #29754, #8422, #58635, #87476, #51498, #80386, #15528, #44403, #37301, #66207, #1323, #30205, #59096, #24023, #81314, #37752, #51970, #74217, #52897, #88874, #89333, #9336, #81776, #32065, #67599, #60496, #73762, #10274, #53848, #59573, #16926, #16460, #68054, #24488, #80860, #30670, #44859, #53368, #10743, #61442, #2268, #88423, #31607, #60037, #45785, #16007, #82714, #82254, #3660, #74697, #17409, #8874, #9819, #3181, #38692, #2727, #17865, #38219, #46257, #75161, #39143, #66660, #31151, #60960, #1787, #89812, #24974, #46717, #23572, #52439, #45312, #75619, #67134, #39600, #68523, #32549, #23088, #26835, #77493, #5999, #85051, #69922, #20200, #61889, #91201, #90721, #12638, #41955, #25882, #70868, #84575, #92149, #76563, #83174, #11686, #48122, #54763, #5062, #27304, #56192, #70415, #83640, #41485, #5540, #26370, #34411, #49079, #34872, #77026, #12154, #55259, #63318, #77978, #18324, #32998, #40999, #69452, #40079, #90272, #18804, #11224, #91684, #76090, #47662, #40537, #55723, #84114, #4582, #13119, #25423, #19723, #19264, #54301, #33457, #62360, #33945, #68996, #62850, #48593, #47180, #4127, #85527, #35809, #43821, #72267, #64268, #36266, #6467, #80283, #71816, #86919, #50476, #36730, #49998, #13575, #22521, #65186, #92615, #73197, #14516, #71337, #289, #27785, #93097, #64723, #72720, #8317, #93550, #7385, #79379, #58065, #44290, #29649, #28708, #65650, #79824, #78439, #21596, #58528, #22072, #49544, #56679, #42902, #764, #43371, #20673, #42425, #29170, #57593, #87373, #50942, #14965, #35344, #7843, #51392, #28251, #6936, #15422, #63785, #86437, #57139, #85980, #21130, #78893, #14040, #30102, #15901, #1218, #58984, #37199, #87832, #22983, #80749, #66107, #44758, #51857, #73658, #20305, #90817, #61982, #76652, #49176, #84206, #4216, #56289, #85152, #70963, #11320, #11777, #13213, #92244, #54397, #25976, #33551, #25518, #32640, #19821, #48215, #19353, #27399, #84670, #18414, #83270, #40629, #63415, #77119, #47274, #90361, #12248, #26465, #78070, #41094, #48687, #76190, #70022, #42049, #40171, #69547, #61530, #69088, #55354, #5165, #33091, #91777, #77591, #55816, #54860, #34508, #83742, #62459, #18899, #47754, #4677, #26928, #91302, #34040, #62943, #12742, #41584, #70506, #5633, #51374, #23898, #58966, #72702, #31023, #59910, #45650, #79806, #80265, #81648, #66997, #29150, #745, #8298, #268, #7365, #88290, #22962, #37180, #23445, #16337, #58047, #43802, #87813, #15401, #50922, #52769, #29629, #22053, #8750, #86898, #36711, #58508, #37629, #66087, #65632, #2134, #88752, #66538, #1200, #16796, #7821, #87353, #15882, #14948, #30082, #22503, #1658, #44738, #44268, #73179, #81190, #73640, #51836, #30537, #80729, #36246, #59439, #52313, #45186, #74089, #9208, #38086, #65164, #47049, #9689, #83988, #25297, #82119, #75950, #38571, #75037, #75490, #83504, #19135, #46591, #18197, #90149, #68865, #55123, #40403, #10614, #47530, #90591, #89209, #89673, #54175, #53236, #24841, #39016, #11082, #61758, #74560, #69321, #83045, #4449, #46134, #39472, #10150, #25751, #26229, #67931, #67473, #3995, #76434, #60828, #2602, #53724, #32412, #3054, #39949, #11555, #33328, #54632, #31939, #18663, #62225, #68390, #91054, #31482, #60370, #61311, #32870, #24360, #82590, #17277, #17737, #3521, #91659, #83146, #39574, #26812, #3631, #18297, #83615, #61415, #90247, #77950, #77000, #54276, #18776, #32971, #63291, #32520, #54737, #25396, #62825, #5036, #47155, #84089, #12611, #4557, #68496, #76064, #40507, #4100, #11193, #40053, #90695, #69426, #11660, #12129, #25855, #33431, #48565, #19239, #40975, #68970, #55698, #70388, #61864, #62335, #47634, #84549, #69897, #76538, #91175, #26341, #33916, #27278, #55234, #48096, #19696, #77468, #41456, #5516, #34386, #92124, #56165, #20174, #85022, #49054, #41931, #71789, #58041, #42876, #64699, #7816, #28226, #43347, #79354, #6911, #27758, #85954, #14489, #70842, #86893, #50452, #35786, #78412, #5975, #20650, #14016, #262, #28684, #93525, #29145, #22047, #34848, #49520, #57570, #21106, #56654, #58502, #35316, #85503, #72244, #92589, #42400, #64241, #7359, #86413, #71311, #72697, #36706, #36241, #21569, #29624, #13551, #6441, #65159, #93072, #50916, #57114, #79800, #14942, #63759, #78866, #43797, #65627, #49974, #739, #87347, #22496, #51369, #13093, #66991, #53230, #66533, #30075, #39011, #52762, #15396, #89667, #31018, #87808, #81643, #44263, #80724, #81185, #89203, #24836 ),
 ( #8293, #59905, #17271, #73174, #88285, #46129, #31933, #74083, #2129, #37174, #45644, #67468, #9684, #73634, #82112, #15877, #16331, #66082, #51831, #30532, #74553, #1194, #44733, #75032, #2597, #67925, #8745, #37622, #59434, #3049, #38080, #1652, #10145, #60824, #80260, #58960, #23440, #22957, #52308, #45181, #9202, #88747, #23893, #16790, #38566, #31477, #60365, #24355, #54171, #83040, #62221, #39469, #54628, #18193, #19131, #91050, #75486, #25747, #33802, #26224, #47045, #55118, #90143, #70277, #61754, #76889, #40398, #26702, #39945, #3517, #12491, #83983, #82586, #63182, #4444, #61307, #47986, #17733, #75946, #83500, #62716, #92013, #18658, #12017, #69316, #40867, #34275, #19587, #47525, #55591, #69785, #68386, #11551, #48456, #4916, #32409, #46588, #32865, #84439, #33324, #10611, #25293, #91546, #76430, #77357, #41343, #5410, #11076, #53719, #68861, #3990, #90586, #57918, #72585, #20998, #13904, #84907, #86307, #14381, #50332, #20544, #29031, #56539, #28120, #48936, #92474, #71203, #21459, #20055, #27640, #86775, #43241, #14835, #85396, #49414, #6330, #43688, #78762, #78304, #50808, #79693, #65505, #5866, #35198, #7707, #21936, #77836, #13443, #57009, #12984, #27165, #72139, #42757, #85845, #7255, #36131, #41822, #63652, #71674, #64126, #70733, #36591, #42291, #34736, #28574, #92961, #49863, #6808, #57464, #35682, #64597, #56053, #93422, #79239, #65048, #151, #80146, #624, #51255, #8177, #15286, #87236, #44143, #22383, #29510, #73047, #37061, #58391, #62806, #76047, #39556, #48548, #62316, #24928, #5496, #40490, #3614, #91156, #53805, #90230, #90679, #5018, #34369, #61848, #33415, #11643, #84070, #70371, #55681, #25839, #91641, #12112, #10699, #47617, #84532, #48078, #75578, #82673, #68953, #26795, #69408, #46675, #17822, #4539, #83596, #19679, #26321, #76983, #68478, #55216, #77449, #32501, #4084, #12593, #41439, #18759, #76520, #61398, #19220, #40957, #69879, #83129, #89766, #25379, #54720, #54259, #18280, #40037, #33899, #47136, #11177, #32955, #50436, #50900, #27740, #92570, #13534, #79784, #21089, #34831, #86877, #22031, #7800, #41912, #42382, #43780, #29127, #85003, #56636, #64224, #56148, #63274, #79339, #78850, #93054, #14474, #72229, #20157, #5957, #49959, #71295, #13076, #14926, #85486, #77933, #64684, #49037, #20633, #49503, #93510, #28210, #78393, #58023, #72681, #28667, #57098, #92107, #63742, #6423, #71774, #14000, #36224, #35298, #70825, #27261, #35771, #85938, #42860, #6897, #57553, #86398, #21552, #43332, #7343, #65143, #244, #8727, #74065, #52289, #31001, #18514, #2579, #66515, #9665, #52743, #51351, #88267, #31458, #88727, #22478, #29607, #15856, #67451, #81168, #87330, #721, #16312, #30516, #60347, #45164, #23875, #58485, #9185, #89184, #80242, #44715, #24337, #83364, #59413, #23423, #15379, #2111, #81624, #59887, #30058, #38548, #66065, #37603, #44243, #8276, #80706, #16772, #73153, #37156, #53212, #45626, #47378, #1177, #58942, #73615, #76292, #38063, #87791, #36687, #65609, #22940, #51813, #1635, #66972, #74533, #90916, #91410, #63046, #76755, #40269, #56399, #27031, #91877, #71068, #6200, #19455, #55920, #84772, #19921, #12850, #63518, #36008, #93295, #80022, #64468, #14255, #64926, #15162, #14715, #43113, #44493, #8507, #44021, #72464, #1408, #79106, #28907, #51139, #28446, #79572, #50686, #72918, #8046, #6678, #43568, #58723, #36939, #29379, #65853, #21332, #30295, #58273, #961, #29840, #87567, #37386, #35555, #22712, #57339, #51586, #80472, #86181, #15622, #66296, #59183, #23185, #78635, #50202, #16547, #66747, #80949, #9426, #81864, #24109, #24575, #38314, #17013, #61057, #2810, #89421, #8962, #39226, #82797, #88510, #45882, #45403, #3265, #53464, #16094, #59667, #73846, #82344, #39687, #90351, #31237, #23657, #60586, #88962, #52990, #44946, #17949, #17492, #32630, #74789, #46344, #37841, #9905, #32155, #38779, #67683, #46800, #67228, #75246, #10361, #31691, #1873, #60123, #68144, #30766, #89899, #25057, #53929, #52523, #81399, #74302, #75703, #2359, #10827, #68612, #3748, #61520, #52067, #12732, #34959, #20295, #5154, #49168, #90808, #26456, #25967, #41574, #70953, #54848, #6085, #19811, #27390, #11768, #18405, #40620, #77108, #83731, #34030, #56280, #85140, #5624, #18890, #70496, #34499, #55345, #63405, #78061, #63871, #12239, #41086, #25507, #47745, #26920, #33542, #48679, #77581, #69079, #54385, #92234, #83261, #4207, #69536, #47264, #76179, #11311, #62934, #40162, #13203, #55807, #33082, #61971, #76643, #91768, #42039, #4669, #62448, #91291, #84659, #84197, #19344, #48206, #70011, #36352, #73285, #21689, #87000, #27875, #57681, #43905, #28794, #50566, #87452, #14134, #29259, #65266, #86524, #13660, #71904, #372, #56768, #72802, #58154, #79463, #64357, #85610, #6557, #93637, #42999, #43454, #71424, #7024, #57225, #22152, #79907, #8398, #22598, #72352, #51473, #93183, #14597, #28335, #15045, #44375, #86066, #37276, #51020, #849, #78981, #20756, #35895, #7469, #21216, #7926, #29730, #58611, #36818, #50086, #65739, #80362, #15503, #92706, #49627, #78523, #42512, #35436, #64813, #30646, #67574, #74192, #89308, #24464, #15983, #66182, #53343, #30181, #44835, #16437, #87913, #23064, #10717, #9794, #80832, #45289, #59546, #89782, #59066, #81291, #51942, #82228, #31584, #73738, #16902, #39118, #31126, #1299, #8850, #67107, #88396, #37728, #66634, #23546, #2241, #38193, #38669, #52416, #60011, #75138, #45761, #2702, #1759, #17382, #3157, #9311, #88851, #24000, #52873, #46234, #81752, #68030, #74670, #60473, #24945, #10249, #32040, #75594, #60935, #53822, #82690, #17840, #46692, #53803, #61846, #62312, #24926, #90228, #68476, #47132, #33413, #18757, #82671, #25837, #68951, #67556, #10697, #47615, #11174, #38652, #45741, #32019, #83594, #3612, #9777, #16882, #32498, #46673, #76518, #61396, #40035, #74652, #25377, #11641, #2685, #60918, #40488, #4537, #75576, #39553, #31565, #18278, #4082, #76045, #46216, #54716, #82210, #17819, #60456, #24444, #3139, #32953, #89291, #53325, #69406, #90677, #91153, #17365, #75120, #89764, #52856, #54257, #10230, #81734, #39098, #68010, #83127, #70369, #8155, #85936, #48076, #19677, #27259, #19218, #65952, #13532, #41910, #56146, #42380, #35295, #76981, #62804, #13074, #5494, #69876, #73027, #48546, #40955, #27738, #12110, #55679, #77446, #56634, #84999, #84530, #21087, #49957, #85484, #20154, #44123, #26793, #12591, #34829, #5015, #49035, #41437, #20631, #63740, #33897, #92105, #6419, #92566, #34367, #49501, #91639, #37038, #26319, #78391, #63272, #77931, #70823, #13996, #84068, #5955, #71293, #64222, #93052, #28208, #57096, #55214, #59768, #39330, #1063, #1983, #59290, #15733, #29942, #52167, #30874, #66848, #67329, #81050, #88609, #10005, #45503, #38420, #51691, #81967, #31793, #37486, #23757, #88136, #45989, #2461, #58827, #8610, #22822, #31337, #82449, #87672, #73946, #66396, #9535, #37939, #52620, #80580, #60687, #60224, #75349, #81502, #89063, #44594, #16649, #74894, #74405, #24213, #89527, #16193, #53088, #17123, #38876, #73498, #9061, #67783, #1512, #2909, #24691, #53574, #30398, #23294, #45045, #17597, #46447, #10464, #46906, #83360, #32732, #4775, #55451, #77697, #63042, #47849, #91873, #39799, #69182, #68721, #84302, #19917, #3851, #48789, #62566, #70134, #54492, #61166 ),
 ( #32260, #18054, #18510, #90002, #25157, #61620, #25609, #69647, #4311, #90452, #34139, #27027, #33657, #62079, #84768, #47374, #76288, #76751, #54031, #33189, #11414, #91407, #11879, #82898, #40265, #48318, #40730, #90912, #26562, #10931, #12846, #26078, #19452, #54967, #41196, #83843, #75807, #55916, #77219, #3372, #68248, #18996, #12347, #5270, #5729, #42146, #42622, #50683, #51136, #13773, #79102, #57335, #36004, #22262, #7580, #71541, #14712, #57792, #56395, #93291, #36465, #25, #27497, #34604, #20863, #72461, #86177, #92342, #63514, #21328, #35551, #65380, #50198, #28904, #85257, #14251, #492, #20405, #49734, #29376, #87112, #64464, #28442, #49275, #7133, #86642, #64922, #35063, #43565, #71064, #6674, #78170, #13308, #85718, #21809, #6196, #63983, #58270, #79569, #80019, #92823, #27986, #78631, #41684, #43109, #56877, #70602, #72016, #53460, #87564, #59180, #89418, #74785, #36936, #8504, #16091, #8042, #15159, #2356, #30762, #44943, #31234, #24106, #65850, #51583, #1870, #88024, #58720, #60583, #37383, #29837, #16544, #958, #73843, #73394, #9902, #38776, #74299, #8959, #31688, #15618, #44490, #23654, #22709, #37838, #66293, #9423, #52520, #80469, #80946, #88959, #81396, #1405, #45400, #30292, #24572, #23181, #38310, #59664, #81861, #52064, #66744, #67680, #67225, #44018, #72915, #88507, #60120, #52987, #17010, #45879, #2806, #61053, #25054, #10358, #3262, #68141, #32152, #82341, #17489, #89896, #46341, #75243, #39223, #35643, #43655, #36095, #63614, #70697, #56971, #14799, #28537, #34700, #41786, #57428, #71636, #72550, #93384, #65015, #5828, #86269, #7672, #92438, #85809, #36555, #29471, #6768, #64560, #27602, #43203, #115, #7221, #71163, #79658, #13407, #78724, #56499, #49375, #28083, #72104, #85358, #78268, #65471, #28996, #588, #42250, #6291, #20959, #58359, #21420, #35161, #87199, #22347, #77798, #20506, #49827, #12948, #64083, #92922, #13865, #42719, #50295, #79201, #86738, #14344, #21900, #50773, #60208, #44107, #87655, #37924, #30381, #1048, #2894, #73482, #65937, #52605, #37023, #80564, #8594, #81487, #9516, #29927, #73011, #59274, #81949, #1967, #8140, #15248, #30859, #45030, #17106, #66829, #38404, #58812, #59753, #45972, #22806, #88120, #74878, #31777, #73930, #88593, #51674, #16634, #67313, #74388, #44579, #53073, #15718, #52152, #37471, #66381, #1497, #45488, #23277, #81034, #9988, #2443, #38861, #16178, #9046, #23742, #67767, #31321, #89047, #60671, #89508, #51219, #24196, #80109, #5255, #84287, #46430, #18039, #25593, #17581, #63028, #11862, #40250, #54476, #40712, #33640, #75333, #61151, #11398, #3836, #68232, #70117, #46891, #39315, #26060, #10449, #54016, #75792, #54949, #83345, #82883, #19437, #48302, #83827, #18492, #41177, #25140, #10914, #33172, #3353, #47356, #39782, #18981, #62062, #32243, #90436, #4759, #90896, #68706, #47833, #89986, #34124, #32718, #76735, #69166, #91392, #61603, #76272, #77202, #69631, #53559, #24673, #4293, #62549, #26547, #82431, #55435, #12332, #7119, #7566, #63965, #35536, #13760, #86162, #72447, #57778, #27972, #64908, #14236, #12832, #49720, #86624, #50186, #41670, #91859, #79084, #55901, #70588, #42132, #19902, #48774, #36451, #64450, #5715, #71049, #85242, #21794, #84754, #13294, #77680, #21314, #57321, #34590, #42608, #10, #56862, #27013, #63498, #92806, #56376, #92328, #27484, #49261, #85704, #20849, #93276, #78156, #78616, #35988, #71524, #28428, #20390, #43095, #28889, #6182, #6658, #35049, #72000, #50669, #79555, #14696, #43551, #37825, #52973, #9889, #44475, #72902, #73832, #8491, #37369, #58255, #31222, #8946, #45865, #88012, #59650, #475, #30276, #16532, #1392, #23166, #60107, #80456, #1858, #66731, #59166, #80004, #73381, #30748, #29363, #45385, #88495, #52049, #36922, #87098, #8026, #66279, #15603, #16078, #44004, #80933, #29823, #23642, #52508, #74771, #88947, #44931, #24094, #65837, #81384, #945, #74286, #16998, #58705, #65366, #9410, #67210, #51570, #22248, #38296, #2343, #87548, #81848, #51118, #15143, #22695, #32141, #83715, #47732, #68597, #18876, #33528, #77095, #90339, #54372, #38764, #3251, #40149, #46786, #61959, #25494, #83247, #67668, #61039, #69065, #75688, #90795, #25954, #82328, #2794, #54835, #31676, #17478, #82783, #60570, #89406, #24560, #76163, #53446, #17935, #89883, #62434, #46329, #53915, #75232, #76631, #4194, #10346, #18393, #11755, #3733, #39212, #68127, #39675, #25043, #10813, #32617, #61507, #47250, #11296, #33069, #40607, #69523, #4654, #91275, #26441, #55332, #84183, #19331, #48193, #70938, #70481, #57207, #13644, #41072, #19797, #34016, #78506, #93619, #50548, #85125, #48666, #20740, #49151, #78047, #5137, #71884, #49611, #86508, #34942, #6541, #69997, #6069, #86048, #42023, #63856, #7006, #27375, #42495, #71409, #92689, #26906, #20276, #35418, #62919, #21197, #64339, #27859, #77567, #91754, #12716, #13188, #56265, #56750, #84646, #85593, #5609, #93166, #28318, #21671, #35878, #50068, #64795, #41558, #78964, #34484, #14115, #57661, #63390, #12225, #42978, #28777, #92220, #55794, #65720, #37261, #15030, #59048, #16420, #45272, #59529, #72785, #30628, #88378, #15488, #23528, #74175, #23983, #9292, #37712, #65249, #72334, #58596, #38175, #30165, #36335, #43438, #87895, #73269, #67090, #1283, #66618, #7453, #23048, #2223, #355, #87437, #31107, #59994, #8381, #66167, #29242, #44819, #1741, #8834, #7910, #81274, #43889, #80346, #58137, #51004, #29714, #73722, #86983, #79891, #88833, #52397, #79445, #36800, #832, #22583, #14581, #51926, #51457, #22136, #44359, #80816, #15965, #26278, #56596, #41876, #4045, #69367, #76944, #68914, #20598, #63237, #91601, #12071, #92068, #84963, #32915, #18713, #62769, #55173, #25800, #27698, #4497, #90637, #77410, #61805, #11604, #33375, #12548, #40919, #40449, #70787, #5922, #41398, #69839, #92532, #76481, #62274, #84495, #54680, #4973, #91109, #70332, #19641, #83554, #48039, #56110, #48509, #84034, #5461, #47576, #85450, #19179, #34331, #26757, #48996, #33859, #55642, #34792, #27222, #11131, #76000, #20114, #77895, #13039, #39995, #63707, #50395, #58452, #58907, #21517, #86838, #65109, #43746, #30024, #15347, #79300, #22442, #65573, #64184, #7311, #93016, #93479, #42821, #73114, #13498, #64650, #6387, #72646, #14892, #71259, #212, #51315, #14440, #87753, #49468, #43297, #13963, #28174, #78358, #6862, #72194, #36190, #21996, #35737, #29092, #87296, #57985, #50868, #35258, #36652, #80207, #85902, #79750, #71736, #687, #7768, #57064, #21054, #49921, #29571, #37121, #78818, #28632, #57521, #44207, #86366, #8241, #66030, #1143, #60312, #3458, #45589, #17212, #51777, #81586, #67871, #52705, #74492, #17681, #38024, #53176, #89150, #16734, #37570, #2071, #24299, #80666, #2994, #82055, #9624, #88227, #15822, #30480, #23839, #66933, #67415, #1597, #30962, #81133, #46073, #10091, #32353, #46533, #2544, #75435, #23383, #38511, #52252, #38959, #68335, #16277, #61252, #74979, #24781, #9146, #44679, #59850, #31423, #45128, #31880, #53663, #82532, #60770, #74029, #89610, #10553, #39418, #22906, #73581, #8690, #66480, #59375, #88691, #54575, #91491, #4394, #19534, #48400, #39887, #90088, #77303, #54114, #68808, #40348, #18137, #46991, #34683, #33745, #3937, #69265, #70679, #55995, #75893, #83446, #90999, #82987, #25240 ),
 ( #90533, #25693, #4862, #11017, #26168, #18601, #55536, #62657, #32811, #62168, #70220, #26646, #47466, #84385, #61701, #12929, #33271, #12435, #76837, #63127, #76373, #11499, #48878, #41285, #55059, #5809, #40812, #83928, #5355, #19080, #47934, #11964, #34221, #69729, #91956, #27111, #84850, #20000, #77781, #41769, #93367, #36539, #79642, #78249, #21402, #29455, #21886, #49355, #56480, #42702, #571, #14327, #20489, #27583, #43187, #57411, #58343, #79183, #50758, #85338, #72088, #87185, #13387, #71620, #22334, #15235, #86251, #50275, #42230, #28980, #14784, #86722, #56954, #65454, #92905, #64541, #71144, #35142, #13849, #57866, #6273, #64065, #51205, #43637, #80093, #28065, #85791, #6753, #44091, #7205, #20942, #72996, #8125, #63597, #72535, #36080, #92421, #49810, #78707, #64998, #35626, #28517, #101, #7654, #45476, #58797, #9034, #17091, #74375, #37457, #9501, #73467, #53546, #45016, #60195, #23729, #9976, #23262, #80546, #89495, #38389, #65923, #46418, #81473, #44564, #67301, #1035, #66366, #37912, #45959, #75319, #66816, #2429, #52592, #31309, #17567, #2881, #1949, #38847, #53061, #51659, #88581, #31766, #89033, #22790, #29913, #16164, #67755, #16621, #87641, #15703, #24182, #30846, #60658, #81936, #74864, #8579, #24658, #82419, #1483, #73917, #37010, #30367, #59739, #59256, #88104, #52140, #81020, #33624, #3823, #12318, #39767, #11385, #32230, #75780, #54461, #69615, #68219, #10900, #70099, #91374, #91844, #68692, #32704, #83332, #26999, #62049, #61590, #34111, #63013, #48759, #82871, #18478, #84740, #5240, #61138, #90422, #40237, #3339, #10436, #26532, #26046, #69152, #55420, #19424, #89974, #46877, #90883, #47340, #54002, #55887, #25579, #25128, #11846, #18024, #76257, #4280, #40696, #33158, #54932, #19888, #39301, #83812, #18965, #47818, #62533, #76720, #4744, #84273, #41162, #48286, #77189, #41656, #28412, #71505, #14678, #93258, #35971, #5698, #57303, #43534, #70573, #85686, #72431, #29342, #6638, #64432, #34573, #43077, #64891, #7100, #71031, #79539, #13278, #78598, #63482, #49245, #27955, #71981, #92312, #78140, #7548, #77959, #65348, #42115, #6164, #56845, #455, #35518, #35034, #36432, #58235, #22228, #56359, #20833, #87079, #77664, #27467, #63948, #13740, #85223, #12816, #28871, #86145, #42590, #57759, #86605, #20374, #92787, #21295, #49702, #50168, #79065, #14217, #21775, #50651, #36899, #80438, #8472, #52489, #80913, #15583, #16979, #45844, #16514, #44911, #67649, #51549, #44454, #59628, #65815, #52028, #73360, #45365, #88475, #72882, #23145, #31203, #23622, #37352, #81364, #87529, #2775, #59147, #74268, #37805, #24075, #66259, #925, #9869, #9391, #79985, #60547, #1840, #58686, #38275, #15122, #1374, #16058, #60088, #89385, #73814, #67188, #66711, #2322, #31656, #74749, #8927, #52951, #88927, #22677, #38744, #51098, #43984, #29805, #30256, #8007, #87992, #30727, #81828, #25474, #17458, #62897, #11736, #40129, #54353, #40589, #33508, #46308, #61018, #11276, #3713, #68106, #69976, #46767, #39194, #25933, #10327, #53896, #75668, #54816, #83227, #82764, #84163, #19311, #83694, #18372, #41049, #25024, #17916, #33048, #3231, #47231, #10792, #18855, #61938, #75212, #90320, #4634, #90774, #39653, #47713, #89864, #5116, #32598, #76613, #69046, #91256, #68576, #32122, #77074, #69503, #53424, #33994, #4175, #61488, #62414, #82308, #76142, #26420, #55310, #24540, #48173, #12205, #13621, #86027, #72311, #57639, #27837, #64773, #14091, #12695, #49589, #86483, #50045, #77545, #84626, #70915, #28756, #42474, #48644, #55773, #71385, #85572, #21648, #6518, #78941, #19774, #35396, #50526, #41535, #6048, #79424, #43416, #20719, #78485, #70461, #57186, #42956, #21176, #85103, #93598, #27354, #92665, #5588, #63368, #42001, #71862, #34460, #92198, #14559, #6983, #7432, #56241, #20253, #34920, #36312, #64316, #49129, #56726, #78025, #35856, #93141, #13165, #63833, #91733, #28296, #26886, #38969, #9156, #82997, #74504, #89621, #53188, #39427, #52716, #16287, #25250, #67881, #1606, #75905, #17222, #74039, #3004, #30491, #66943, #67426, #75444, #11030, #38522, #10102, #82066, #60781, #47002, #32363, #2554, #68344, #82541, #81143, #24309, #61264, #24789, #52263, #59386, #45602, #3471, #46084, #23397, #88238, #74991, #60322, #90099, #31890, #53674, #45138, #17692, #54126, #38036, #9634, #18148, #65228, #89160, #46542, #2083, #10563, #30973, #59861, #88702, #23850, #81597, #31433, #16747, #11511, #83938, #5366, #3950, #40358, #5820, #27123, #27596, #4404, #69275, #19091, #56493, #91501, #33283, #63608, #92432, #78262, #18613, #47945, #20500, #34694, #61712, #62178, #40822, #32822, #39898, #56006, #55546, #69741, #84862, #48891, #90546, #76385, #26657, #76847, #83458, #85352, #91010, #54586, #41296, #25704, #26179, #55069, #70231, #4873, #11974, #49368, #68820, #34232, #33756, #47477, #62668, #84396, #48411, #19545, #77314, #12448, #63138, #91967, #20013, #77792, #12941, #41780, #70690, #58355, #43199, #65010, #8135, #28531, #43650, #79654, #7217, #28078, #86264, #14795, #42243, #87195, #50769, #36090, #78719, #6285, #20954, #14340, #57424, #57878, #85803, #21415, #71632, #72546, #583, #22802, #37018, #86733, #65932, #13860, #72100, #42715, #29466, #58807, #6764, #87651, #7667, #15244, #93380, #35156, #50290, #111, #35638, #21896, #44101, #73007, #22343, #64556, #51214, #80105, #28990, #1044, #29923, #51669, #36550, #65466, #13399, #79197, #71156, #64077, #92916, #56966, #49822, #80559, #59268, #15713, #73477, #66376, #44574, #37467, #8589, #1493, #88116, #23273, #30377, #81630, #22037, #73160, #14932, #81173, #23428, #50906, #8733, #31006, #22946, #2584, #58029, #58949, #22484, #72687, #86883, #15385, #87797, #30064, #30520, #44250, #51820, #66978, #37609, #1640, #43787, #45169, #88733, #727, #80712, #51358, #9190, #59419, #79790, #65615, #7806, #88272, #45631, #36694, #37162, #29613, #66521, #66071, #52295, #58491, #38068, #16317, #15863, #87336, #80249, #8282, #44721, #1183, #74071, #73621, #2116, #59892, #23880, #52748, #67456, #16777, #74539, #9670, #38553, #32397, #31919, #47513, #76880, #60811, #12007, #25735, #33314, #17721, #24342, #46576, #83028, #89653, #11063, #62210, #91040, #11541, #24822, #76419, #40388, #61296, #69306, #26212, #69775, #18182, #47033, #60352, #53706, #32854, #39458, #54617, #83489, #75019, #89189, #18646, #53217, #10132, #75474, #82098, #17257, #46116, #68850, #38998, #10598, #82573, #55106, #67911, #68375, #3036, #4434, #90575, #3505, #75935, #83973, #90131, #25282, #54159, #39933, #3979, #61743, #19121, #47976, #40857, #70724, #71193, #56043, #34727, #13894, #49405, #42280, #55581, #85836, #35672, #41331, #63643, #63172, #49854, #6320, #33790, #12481, #26692, #35188, #86297, #43231, #77825, #70266, #13433, #41813, #5856, #91535, #64587, #64113, #79229, #27630, #92951, #62705, #92465, #78753, #56529, #85386, #93412, #20046, #28111, #56998, #20535, #19577, #78295, #28564, #84429, #12975, #57455, #50323, #20987, #42748, #48445, #71664, #6797, #21450, #92002, #14371, #34265, #4905, #77347, #5400, #48926, #27155, #84896, #73849, #39231, #60589, #61060, #37844, #8966, #23661, #89902, #31240, #44949, #3268, #32159, #17952, #52070, #52527, #53932, #68148, #1412, #66750, #74305, #66298, #73400, #89424, #88966, #9430, #24579, #82347 ),
 ( #38317, #1877, #53467, #25060, #30770, #82801, #67686, #75249, #59670, #30299, #88513, #60127, #81402, #52993, #10364, #8510, #17495, #16551, #46348, #37389, #67232, #59186, #88031, #23188, #24113, #81867, #80953, #45406, #74792, #2362, #2814, #31696, #16097, #17017, #45886, #9909, #38782, #90810, #68616, #3751, #85144, #84199, #61523, #25969, #40165, #70499, #10830, #61975, #32633, #70014, #12241, #39691, #91295, #19814, #11770, #90354, #54852, #69081, #5626, #25511, #83734, #54389, #5157, #41088, #83263, #26458, #48681, #40623, #46804, #75707, #47747, #11313, #18408, #47266, #4209, #76645, #18892, #19346, #33084, #69539, #55809, #55347, #48208, #76182, #34033, #77583, #4671, #33544, #62451, #91770, #77111, #62936, #26922, #84662, #12734, #34501, #41577, #63408, #92237, #27392, #56282, #86070, #13206, #79911, #57684, #852, #43003, #14600, #49170, #78984, #65270, #50090, #71907, #15048, #35440, #50570, #86527, #14138, #34961, #93186, #21693, #78063, #375, #79466, #7028, #85613, #42041, #27880, #21220, #64361, #64816, #92710, #28338, #78526, #43458, #7472, #29733, #43909, #93640, #72805, #20759, #35898, #49631, #36357, #65743, #13664, #58614, #72355, #22155, #6561, #70956, #57228, #28799, #42516, #29263, #51023, #7930, #58158, #71427, #87003, #36823, #20298, #6088, #63873, #56771, #45292, #9314, #87455, #51945, #88854, #1765, #16906, #45764, #37279, #22602, #74674, #51477, #66185, #37731, #15506, #44379, #32044, #31129, #44838, #24003, #23550, #80837, #53347, #82231, #52876, #81294, #10253, #87916, #23067, #2245, #73289, #88400, #15986, #81755, #60015, #8401, #59549, #67577, #9798, #73741, #38672, #30184, #39121, #30649, #2705, #74196, #60476, #8853, #1302, #46237, #31587, #80365, #3160, #38197, #59072, #89312, #66638, #52419, #16440, #24467, #67110, #17388, #75141, #68033, #55238, #41460, #26817, #90698, #33920, #77005, #75597, #18779, #55703, #19243, #46695, #53827, #40057, #91663, #11664, #17844, #24950, #40513, #54740, #84554, #76541, #48102, #82693, #69431, #19701, #10720, #68974, #48571, #12615, #83618, #47638, #39577, #26345, #12134, #84094, #54279, #62829, #90251, #61867, #68500, #32525, #11197, #40979, #3634, #61419, #77472, #69901, #70392, #25400, #83149, #4104, #5520, #4561, #18300, #60938, #89786, #47158, #76067, #32976, #25858, #33435, #62339, #91179, #5040, #27283, #72701, #21574, #49978, #64246, #50456, #43352, #56170, #70847, #21110, #13555, #77954, #79805, #56658, #49058, #35790, #20178, #63764, #86417, #85027, #14020, #65163, #92128, #42405, #267, #14947, #28230, #78871, #13097, #93530, #79359, #57574, #27763, #36245, #92594, #35321, #41935, #5980, #78417, #28688, #34852, #85507, #29149, #14494, #22052, #20654, #49524, #71315, #50921, #85959, #6446, #58046, #86897, #34390, #93076, #57118, #43801, #63297, #42881, #71794, #6916, #64703, #72248, #7364, #23444, #37628, #88751, #16795, #744, #44267, #88289, #80728, #51373, #53235, #30081, #22502, #9207, #87352, #37179, #58965, #38085, #66537, #66086, #67472, #2601, #66996, #1657, #24359, #8297, #1199, #16336, #80264, #8749, #87812, #2133, #45185, #29628, #73639, #81647, #74088, #22961, #31022, #73178, #82118, #15881, #59909, #52312, #74559, #51835, #15400, #60369, #23897, #36710, #17276, #81189, #44737, #52768, #65631, #30536, #59438, #45649, #46133, #9688, #38570, #31481, #89208, #7820, #58507, #31938, #53723, #24840, #10149, #60827, #82589, #17736, #39015, #75036, #89672, #67930, #3053, #27382, #34490, #21205, #64347, #7459, #86055, #6075, #71415, #92226, #42030, #20746, #35885, #63396, #70944, #36341, #57670, #58143, #34949, #63862, #49617, #86989, #28325, #92695, #362, #29248, #15035, #49158, #78513, #51010, #65256, #56271, #27865, #6547, #85131, #70487, #86515, #50076, #35425, #21678, #79451, #20283, #13194, #57214, #13650, #78053, #22142, #56757, #85599, #71892, #42502, #93173, #78971, #7013, #14122, #42986, #79897, #5616, #64802, #93626, #28784, #50554, #14587, #43444, #72340, #44825, #73276, #9300, #52405, #65727, #15972, #23990, #81281, #44365, #16427, #80353, #60463, #51932, #67097, #30636, #16891, #30171, #87443, #2692, #45279, #72792, #53332, #88385, #51464, #74182, #7916, #8388, #73728, #52863, #82218, #8840, #38182, #59535, #2231, #24453, #9784, #37718, #45748, #60001, #58602, #1748, #38659, #31114, #29720, #36807, #23054, #74660, #23535, #838, #22589, #88841, #66624, #67563, #81741, #31574, #15494, #89298, #43895, #37267, #80822, #66173, #1289, #59054, #87902, #75128, #76527, #4546, #40497, #10706, #19227, #54726, #32029, #61405, #39563, #40963, #10238, #32508, #68019, #69415, #11650, #39106, #61854, #84077, #76053, #55687, #17372, #18287, #75585, #60926, #46224, #68485, #47144, #83136, #83603, #3621, #11183, #26329, #90685, #18766, #3147, #33421, #48085, #53812, #40043, #90237, #62323, #47624, #89773, #24935, #82680, #91163, #5024, #17830, #25386, #46682, #25845, #54266, #68959, #4090, #76989, #55223, #91647, #32961, #12118, #69885, #33905, #62813, #26801, #42388, #79345, #5963, #21096, #57104, #78400, #5503, #63748, #85944, #19685, #64690, #28216, #13540, #56154, #77455, #92113, #85492, #34837, #35304, #63280, #92577, #49043, #49965, #71780, #251, #14480, #64230, #43338, #85010, #20639, #20163, #6902, #36231, #77938, #65149, #78856, #86404, #70831, #12599, #27746, #71300, #13082, #93060, #21558, #50442, #93516, #41919, #35777, #28674, #49509, #57560, #72235, #29134, #6429, #14006, #84538, #56642, #42866, #7349, #48554, #41445, #34375, #70377, #27267, #66257, #52024, #52486, #30254, #59145, #46764, #81361, #25021, #60085, #73811, #32119, #61015, #8470, #80910, #16511, #82761, #68103, #87989, #1837, #9388, #1372, #37350, #89382, #24072, #38272, #24537, #17455, #23142, #44908, #88924, #45362, #16055, #53893, #30724, #8924, #9866, #37802, #66708, #59624, #38741, #67184, #88472, #3228, #89861, #67646, #2319, #17913, #23619, #74265, #16976, #31200, #52948, #81825, #2772, #45841, #74745, #60544, #82304, #53421, #46305, #75209, #10324, #39191, #83691, #5113, #62411, #48640, #61935, #25471, #34456, #48170, #10789, #85100, #26417, #83224, #77071, #39650, #76139, #76609, #84623, #20250, #47710, #19308, #91253, #69973, #56237, #41532, #11733, #77542, #91730, #90317, #33504, #70458, #33991, #61485, #68573, #54813, #12692, #55307, #32595, #3710, #84160, #69500, #5585, #12202, #62894, #54350, #41045, #63365, #18369, #18852, #92195, #27351, #4631, #26883, #47229, #55770, #19771, #75665, #69043, #11273, #40126, #40586, #4172, #33045, #25930, #90771, #13162, #49586, #15006, #36309, #36774, #13618, #78482, #58114, #78937, #29215, #43865, #87412, #6980, #64770, #49126, #42471, #50523, #57183, #72308, #7429, #92662, #78022, #65225, #41998, #27834, #93138, #70912, #6045, #34917, #86479, #63829, #28293, #71381, #72762, #56723, #64313, #85569, #329, #14556, #20716, #93595, #22112, #14088, #6515, #35393, #50042, #86024, #21173, #42953, #71859, #35853, #28753, #21645, #57636, #79421, #86959, #43413, #50981, #79866, #7883, #65694, #808, #29688, #58572, #67530, #23954, #51433, #30141, #44334, #88807, #10204, #60887, #1715, #59025, #31081, #59501, #88353, #15461, #82183, #59969, #3112, #45245, #16856, #80322, #81247, #2660, #52372, #74150, #17339, #37688, #52829, #81707, #16394, #37239 ) ),
 .UNSPECIFIED., .F., .F., .F.,
 ( 4, 3, 3, 3, 3, 3, 3, 3, 3, 3, 3, 3, 4 ),
 ( 4, 3, 3, 3, 3, 3, 3, 3, 3, 3, 3, 3, 3, 3, 3, 3, 3, 3, 3, 3, 3, 3, 3, 3, 3, 3, 3, 3, 3, 3, 3, 3, 3, 3, 3, 3, 3, 3, 3, 3, 3, 3, 3, 3, 3, 3, 3, 3, 3, 3, 3, 3, 3, 3, 3, 3, 3, 3, 3, 3, 3, 3, 3, 3, 3, 3, 3, 3, 3, 3, 3, 3, 3, 3, 3, 3, 3, 3, 3, 3, 3, 3, 3, 3, 3, 3, 3, 3, 3, 3, 3, 3, 3, 3, 3, 3, 3, 3, 3, 3, 3, 3, 3, 3, 3, 3, 3, 3, 3, 3, 3, 3, 3, 3, 3, 3, 3, 3, 3, 3, 3, 3, 3, 3, 3, 3, 3, 3, 3, 3, 3, 3, 3, 3, 3, 3, 3, 3, 3, 3, 3, 3, 3, 3, 3, 3, 3, 3, 3, 3, 3, 3, 3, 3, 3, 3, 3, 3, 3, 3, 3, 3, 3, 3, 3, 3, 3, 3, 3, 3, 3, 3, 3, 3, 3, 3, 3, 3, 3, 3, 3, 3, 3, 3, 3, 3, 3, 3, 3, 3, 3, 3, 3, 3, 3, 3, 3, 3, 3, 3, 3, 3, 3, 3, 3, 3, 3, 3, 3, 3, 3, 3, 3, 3, 3, 3, 3, 3, 3, 3, 3, 3, 3, 3, 3, 3, 3, 3, 3, 3, 3, 3, 3, 3, 3, 3, 3, 3, 3, 3, 3, 3, 3, 3, 3, 3, 3, 3, 3, 3, 3, 3, 3, 3, 3, 3, 3, 3, 3, 3, 3, 3, 3, 3, 3, 3, 3, 3, 3, 3, 3, 3, 3, 3, 3, 3, 3, 3, 3, 3, 3, 3, 3, 3, 3, 3, 3, 3, 3, 3, 3, 3, 3, 3, 3, 3, 3, 3, 3, 3, 3, 3, 3, 4 ),
 ( -1.998401444325281773E-15, 0.06249999999999825140, 0.1249999999999985012, 0.1562499999999986122, 0.1874999999999987510, 0.2187499999999988898, 0.2499999999999990008, 0.2812499999999991118, 0.3124999999999992228, 0.3437499999999993339, 0.3749999999999995004, 0.4374999999999997780, 0.5000000000000000000 ),
 ( -0.05654842365434873536, -0.02821878541515033395, -0.01405396629555113498, -0.006971556735751535498, -0.003430351955851735756, -0.001659749565901835885, -0.0007744483709268859496, -0.0003317977734394109818, 0.0001108528240480639859, 0.003652057603947863728, 0.007193262383847663470, 0.01073446716374746278, 0.01427567194364726295, 0.01781687672354706140, 0.02135808150344686157, 0.02489928628334666175, 0.02844049106324646192, 0.03021109345319636375, 0.03198169584314626557, 0.03552290062304606227, 0.03906410540294585898, 0.04260531018284566263, 0.04437591257279556445, 0.04614651496274546627, 0.04968771974264526298, 0.05322892452254505968, 0.05677012930244486333, 0.05854073169239476515, 0.06031133408234466003, 0.06385253886224445674, 0.06739374364214426039, 0.07093494842204406403, 0.07270555081199396585, 0.07447615320194386768, 0.07801735798184365744, 0.08155856276174344721, 0.08509976754164325086, 0.08687036993159315268, 0.08864097232154305450, 0.09218217710144285815, 0.09572338188134266179, 0.09926458666124245156, 0.1010351890511923534, 0.1028057914411422413, 0.1063469962210420450, 0.1098882010009418486, 0.1134294057808416523, 0.1152000081707915541, 0.1169706105607414559, 0.1205118153406412596, 0.1240530201205410632, 0.1275942249004408668, 0.1293648272903907825, 0.1311354296803406705, 0.1346766344602404741, 0.1382178392401402500, 0.1417590440200400537, 0.1435296464099899416, 0.1453002487999398573, 0.1488414535798396332, 0.1523826583597394368, 0.1559238631396392405, 0.1576944655295891562, 0.1594650679195390441, 0.1630062726994388478, 0.1665474774793386514, 0.1700886822592384551, 0.1718592846491883708, 0.1736298870391382587, 0.1771710918190380624, 0.1807122965989378660, 0.1842535013788376697, 0.1860241037687875854, 0.1877947061587374733, 0.1913359109386372769, 0.1948771157185370528, 0.1984183204984368565, 0.2001889228883867444, 0.2019595252783366601, 0.2055007300582364360, 0.2090419348381362397, 0.2125831396180360433, 0.2143537420079859590, 0.2161243443979358470, 0.2196655491778356506, 0.2232067539577354542, 0.2267479587376352579, 0.2285185611275851736, 0.2302891635175350615, 0.2338303682974348652, 0.2373715730773346411, 0.2409127778572344447, 0.2426833802471843327, 0.2444539826371342484, 0.2479951874170340242, 0.2515363921969338001, 0.2550775969768336315, 0.2568481993667835472, 0.2586188017567334629, 0.2621600065366332388, 0.2657012113165330147, 0.2692424160964328461, 0.2710130184863827618, 0.2727836208763326775, 0.2763248256562324534, 0.2798660304361322293, 0.2834072352160320607, 0.2851778376059819764, 0.2869484399959318921, 0.2904896447758316680, 0.2940308495557314439, 0.2975720543356312753, 0.2993426567255811910, 0.3011132591155311067, 0.3046544638954308826, 0.3081956686753306585, 0.3117368734552304899, 0.3135074758451804056, 0.3152780782351303213, 0.3188192830150300972, 0.3223604877949298730, 0.3259016925748297044, 0.3276722949647795646, 0.3294428973547294803, 0.3329841021346292562, 0.3365253069145290876, 0.3400665116944288635, 0.3418371140843787792, 0.3436077164743286394, 0.3471489212542284708, 0.3506901260341282467, 0.3542313308140280226, 0.3560019332039779383, 0.3577725355939278540, 0.3613137403738276299, 0.3648549451537274058, 0.3683961499336272372, 0.3701667523235771529, 0.3719373547135270686, 0.3754785594934268445, 0.3790197642733266203, 0.3825609690532264517, 0.3843315714431763674, 0.3861021738331262831, 0.3896433786130260590, 0.3931845833929258349, 0.3967257881728256663, 0.3984963905627755820, 0.4002669929527254977, 0.4038081977326252736, 0.4073494025125250495, 0.4108906072924248809, 0.4126612096823747966, 0.4144318120723247123, 0.4179730168522244882, 0.4215142216321242641, 0.4250554264120240955, 0.4285966311919239269, 0.4321378359718237028, 0.4356790407517234787, 0.4392202455316233101, 0.4427614503115230860, 0.4463026550914228618, 0.4498438598713226932, 0.4533850646512224691, 0.4569262694311222450, 0.4586968718210721607, 0.4604674742110220764, 0.4640086789909218523, 0.4675498837708216282, 0.4710910885507214596, 0.4728616909406713198, 0.4746322933306212355, 0.4781734981105210114, 0.4817147028904208428, 0.4852559076703206742, 0.4870265100602705344, 0.4887971124502204501, 0.4923383172301202260, 0.4958795220100200574, 0.4994207267899198888, 0.5011913291798697490, 0.5029619315698197202, 0.5065031363497194405, 0.5100443411296192719, 0.5135855459095191033, 0.5153561482994689635, 0.5171267506894188237, 0.5206679554693186551, 0.5242091602492184865, 0.5277503650291182069, 0.5295209674190681781, 0.5312915698090180383, 0.5348327745889178697, 0.5383739793688175901, 0.5419151841487174215, 0.5436857865386672817, 0.5454563889286172529, 0.5489975937085169733, 0.5525387984884168047, 0.5560800032683166361, 0.5578506056582664963, 0.5596212080482163564, 0.5631624128281161878, 0.5667036176080160192, 0.5702448223879158506, 0.5720154247778657108, 0.5737860271678156820, 0.5773272319477154024, 0.5808684367276152338, 0.5844096415075150652, 0.5861802438974649254, 0.5879508462874147856, 0.5914920510673146170, 0.5950332558472144484, 0.5985744606271142798, 0.6003450630170641400, 0.6021156654070141112, 0.6056568701869138316, 0.6091980749668136630, 0.6127392797467134944, 0.6145098821366633546, 0.6162804845266132148, 0.6198216893065130462, 0.6233628940864128776, 0.6269040988663127090, 0.6286747012562625692, 0.6304453036462125404, 0.6339865084261122608, 0.6375277132060120922, 0.6410689179859119236, 0.6428395203758617837, 0.6446101227658116439, 0.6481513275457114753, 0.6516925323256113067, 0.6552337371055111381, 0.6570043394954609983, 0.6587749418854109695, 0.6623161466653106899, 0.6658573514452105213, 0.6693985562251103527, 0.6711691586150602129, 0.6729397610050100731, 0.6764809657849099045, 0.6800221705648097359, 0.6835633753447095673, 0.6853339777346594275, 0.6871045801246093987, 0.6906457849045091191, 0.6941869896844089505, 0.6977281944643087819, 0.6994987968542586421, 0.7012693992442085023, 0.7048106040241083337, 0.7083518088040081651, 0.7118930135839078854, 0.7136636159738578566, 0.7154342183638077168, 0.7189754231437075482, 0.7225166279236072686, 0.7260578327035071000, 0.7278284350934569602, 0.7295990374834069314, 0.7331402422633066518, 0.7366814470432064832, 0.7402226518231063146, 0.7419932542130561748, 0.7437638566030060350, 0.7473050613829058664, 0.7508462661628056978, 0.7543874709427054182, 0.7561580733326553894, 0.7579286757226052496, 0.7614698805025050810, 0.7650110852824048013, 0.7685522900623046327, 0.7703228924522544929, 0.7720934948422044641, 0.7756346996221041845, 0.7791759044020040159, 0.7827171091819038473, 0.7844877115718537075, 0.7862583139618035677, 0.7897995187417033991, 0.7933407235216032305, 0.7968819283015030619, 0.7986525306914529221, 0.8004231330814028933, 0.8039643378613026137, 0.8075055426412024451, 0.8110467474211022765, 0.8128173498110521367, 0.8145879522010019969, 0.8181291569809018283, 0.8216703617608016597, 0.8252115665407014911, 0.8269821689306513512, 0.8287527713206013225, 0.8322939761005010428, 0.8358351808804008742, 0.8393763856603007056, 0.8429175904402004260, 0.8464587952201002574, 0.8500000000000000888 ),
 .UNSPECIFIED. ) ;
#54165=CARTESIAN_POINT ( 'NONE',  ( -15.81668226956704437, -284.5299966992748182, -341.1752946549420926 ) ) ;
#54166=CARTESIAN_POINT ( 'NONE',  ( -99.56188087693280409, -292.5693872661504997, -226.0073650280881452 ) ) ;
#54167=CARTESIAN_POINT ( 'NONE',  ( -22.30719664980588490, -293.5558465555933481, -195.2920634523905790 ) ) ;
#54168=CARTESIAN_POINT ( 'NONE',  ( 16.15769396357575616, -294.0993445966775539, -320.0281577205441295 ) ) ;
#54169=CARTESIAN_POINT ( 'NONE',  ( 17.41777575143020229, -288.8344578622092627, -219.0937542781570926 ) ) ;
#54170=CARTESIAN_POINT ( 'NONE',  ( 11.49423899803039006, -282.5632069539214513, -329.9620495350150691 ) ) ;
#54171=CARTESIAN_POINT ( 'NONE',  ( -96.20880343660680012, -295.2789984273261439, -222.9904693623223011 ) ) ;
#54172=CARTESIAN_POINT ( 'NONE',  ( 9.207117593550204759, -282.2657466507333766, -331.6979549828733980 ) ) ;
#54173=CARTESIAN_POINT ( 'NONE',  ( 36.33469206697079557, -277.6906994140549614, -282.6588970334490796 ) ) ;
#54174=CARTESIAN_POINT ( 'NONE',  ( -67.68488546085839630, -297.9805209788416391, -333.4427485647536855 ) ) ;
#54175=CARTESIAN_POINT ( 'NONE',  ( -96.11153733409877020, -276.0394692712719689, -318.1978790994803035 ) ) ;
#54177=CARTESIAN_POINT ( 'NONE',  ( -91.71503398925338502, -283.3617779264020555, -319.1808570932154225 ) ) ;
#54178=CARTESIAN_POINT ( 'NONE',  ( -7.704856378814294970, -281.6371007568332061, -199.7093206184912901 ) ) ;
#54179=CARTESIAN_POINT ( 'NONE',  ( 28.50291222047669493, -286.0935370845697321, -230.7958420713842997 ) ) ;
#54180=CARTESIAN_POINT ( 'NONE',  ( -60.59835322099827692, -293.5065951240130175, -200.0428200160021959 ) ) ;
#54181=CARTESIAN_POINT ( 'NONE',  ( 35.30614460431431922, -277.4443150188960203, -293.3552709575204744 ) ) ;
#54182=CARTESIAN_POINT ( 'NONE',  ( 21.46101486130531555, -276.2047420173916521, -221.4168743546945848 ) ) ;
#54183=CARTESIAN_POINT ( 'NONE',  ( -45.91020518985178711, -276.9970026567052628, -342.9071279572621052 ) ) ;
#54184=CARTESIAN_POINT ( 'NONE',  ( -76.18347497306811533, -299.5323573762630645, -206.3374066044498534 ) ) ;
#54185=CARTESIAN_POINT ( 'NONE',  ( -44.16684723920729283, -283.9654691774103981, -195.8396727926966037 ) ) ;
#54186=CARTESIAN_POINT ( 'NONE',  ( -22.19379459336163407, -291.9076566441407294, -194.8330674582151971 ) ) ;
#54187=CARTESIAN_POINT ( 'NONE',  ( -110.4702084345482973, -292.4237138758828110, -248.9447296573441122 ) ) ;
#54188=CARTESIAN_POINT ( 'NONE',  ( -1.091915261902661749, -291.4656311383803313, -206.6270448332325032 ) ) ;
#54190=CARTESIAN_POINT ( 'NONE',  ( 6.175662656369911296, -291.2049992168653034, -207.5531134937818933 ) ) ;
#54192=CARTESIAN_POINT ( 'NONE',  ( -46.99305993686557770, -291.5928996371412154, -197.9806044408231287 ) ) ;
#54194=CARTESIAN_POINT ( 'NONE',  ( -91.37096054294096348, -290.8784016147202465, -324.8631133841032010 ) ) ;
#54195=CARTESIAN_POINT ( 'NONE',  ( -94.87621839796359779, -279.8387046437596837, -225.2447159202324656 ) ) ;
#54196=CARTESIAN_POINT ( 'NONE',  ( -111.9703692608760548, -295.6943165506294804, -252.6960605321189632 ) ) ;
#54197=CARTESIAN_POINT ( 'NONE',  ( -73.57233305379359933, -286.2360350986262461, -202.4740180238676999 ) ) ;
#54198=CARTESIAN_POINT ( 'NONE',  ( 14.22956605511410899, -287.0863711728291605, -213.1393770527902234 ) ) ;
#54199=CIRCLE ( 'NONE', #63296, 5.841085083515828558 ) ;
#54200=CARTESIAN_POINT ( 'NONE',  ( -109.5185953549989364, -284.7351460723400010, -281.7571326386113242 ) ) ;
#54201=CARTESIAN_POINT ( 'NONE',  ( -48.55409767855074676, -154.7049544282185707, -365.0407483515538161 ) ) ;
#54202=CARTESIAN_POINT ( 'NONE',  ( 4.175116275386621112, -57.89727328217816194, -353.1401067649683228 ) ) ;
#54203=CARTESIAN_POINT ( 'NONE',  ( -13.16113611277997286, -92.07136048423980412, -356.2614093299528690 ) ) ;
#54204=CARTESIAN_POINT ( 'NONE',  ( -16.34428335865657544, -275.9710053673329639, -340.4978363436782729 ) ) ;
#54205=CARTESIAN_POINT ( 'NONE',  ( -26.99140282775333333, -275.8377754050243880, -342.9358892107668453 ) ) ;
#54206=CARTESIAN_POINT ( 'NONE',  ( -80.58524852322130982, -296.9908841998434923, -206.6612070728645847 ) ) ;
#54207=CARTESIAN_POINT ( 'NONE',  ( -101.2730542070560631, -255.2172494999240939, -324.5853935562917059 ) ) ;
#54208=CARTESIAN_POINT ( 'NONE',  ( -17.50202521352245100, -275.4861885082246431, -344.2508031272387825 ) ) ;
#54209=CARTESIAN_POINT ( 'NONE',  ( -104.1289863278719992, -274.7377560944700576, -238.4639016002249150 ) ) ;
#54210=CARTESIAN_POINT ( 'NONE',  ( -107.0622175921625541, -291.3342242559098736, -248.4777640785070787 ) ) ;
#54211=CARTESIAN_POINT ( 'NONE',  ( -66.85294953455573363, -296.2319582254946226, -341.3206550665373697 ) ) ;
#54212=CARTESIAN_POINT ( 'NONE',  ( -40.44406008143359799, -298.5066111514885847, -193.4331447318857897 ) ) ;
#54213=CARTESIAN_POINT ( 'NONE',  ( -6.762974776336586835, -294.8058561910875710, -336.6479308520583800 ) ) ;
#54215=CARTESIAN_POINT ( 'NONE',  ( -45.46994408713371882, -279.0743969435646932, -345.5347241672198493 ) ) ;
#54216=ADVANCED_FACE ( 'NONE', ( #53349 ), #16741, .T. ) ;
#54217=CARTESIAN_POINT ( 'NONE',  ( -1.158829664570814266, -280.0268634296121490, -202.4617307364441388 ) ) ;
#54218=CARTESIAN_POINT ( 'NONE',  ( -4.951263143486116292, -277.5561718139133518, -336.0581420091110090 ) ) ;
#54219=CARTESIAN_POINT ( 'NONE',  ( 38.69364737444505664, -277.3221468995234886, -271.1386050336082008 ) ) ;
#54220=CARTESIAN_POINT ( 'NONE',  ( -106.0557790435301371, -271.3861665340733680, -243.5918377119631089 ) ) ;
#54223=CARTESIAN_POINT ( 'NONE',  ( -103.3707550275782125, -279.1408952144284399, -239.1108996205265953 ) ) ;
#54224=CARTESIAN_POINT ( 'NONE',  ( -0.1326142521014597453, -275.3369914631144297, -203.1178688480154904 ) ) ;
#54225=CARTESIAN_POINT ( 'NONE',  ( -34.70072416815290239, -287.7044471030052364, -346.8223730069888120 ) ) ;
#54226=CARTESIAN_POINT ( 'NONE',  ( -19.06272597346500675, -276.2874411237381196, -197.5690879805409566 ) ) ;
#54228=CARTESIAN_POINT ( 'NONE',  ( -104.1994306258546459, -289.3487598654411386, -300.1956215619385375 ) ) ;
#54229=CARTESIAN_POINT ( 'NONE',  ( -83.20842201836086360, -284.7912459432007495, -208.5731160702488580 ) ) ;
#54230=CARTESIAN_POINT ( 'NONE',  ( 33.71362441991469439, -279.5217295442126897, -249.6460300550033651 ) ) ;
#54231=CARTESIAN_POINT ( 'NONE',  ( 33.52199464820392194, -280.3870375958060777, -290.2032872373982286 ) ) ;
#54232=CARTESIAN_POINT ( 'NONE',  ( -24.87709350065013325, -284.2920719180544324, -196.9197892110969974 ) ) ;
#54233=CARTESIAN_POINT ( 'NONE',  ( -72.52723074908284673, -291.5180280395061914, -336.6096410231270397 ) ) ;
#54234=CARTESIAN_POINT ( 'NONE',  ( -109.2794766816137866, -279.9491332198462601, -255.7347404808160718 ) ) ;
#54236=CARTESIAN_POINT ( 'NONE',  ( 3.411515403631638854, -278.9897245405375656, -205.9123239624678661 ) ) ;
#54237=CARTESIAN_POINT ( 'NONE',  ( -25.36654160979586692, -294.2049700471081337, -196.3233153089201721 ) ) ;
#54238=CARTESIAN_POINT ( 'NONE',  ( -111.0968542681884514, -277.0243621970629988, -252.0279950036088508 ) ) ;
#54239=CARTESIAN_POINT ( 'NONE',  ( -21.62302894800675901, -277.4968351821499368, -341.8051730164002038 ) ) ;
#54240=CARTESIAN_POINT ( 'NONE',  ( -19.33235961746500564, -284.8212877188626067, -343.3921109489503465 ) ) ;
#54242=CARTESIAN_POINT ( 'NONE',  ( -111.4507632717454442, -292.2836565199086181, -285.1629776817619017 ) ) ;
#54243=CARTESIAN_POINT ( 'NONE',  ( 28.56531585670742146, -286.2319341979917908, -230.7562762363980085 ) ) ;
#54244=CARTESIAN_POINT ( 'NONE',  ( -33.44604961925815445, -290.5018405187756230, -196.6513770150382072 ) ) ;
#54246=CARTESIAN_POINT ( 'NONE',  ( 24.38957341470759133, -274.7865101104688392, -310.3359109574766990 ) ) ;
#54247=CARTESIAN_POINT ( 'NONE',  ( 29.49653226403537332, -292.1230395086887484, -302.7830874750350745 ) ) ;
#54250=CARTESIAN_POINT ( 'NONE',  ( -96.91006988601124306, -289.6766801822311663, -222.6713173928956735 ) ) ;
#54251=CARTESIAN_POINT ( 'NONE',  ( -44.11789767307843846, -287.5651773448868767, -196.8728633981021403 ) ) ;
#54252=CARTESIAN_POINT ( 'NONE',  ( -3.532012552953720963, -286.8519857654526390, -338.4261147132313567 ) ) ;
#54253=CARTESIAN_POINT ( 'NONE',  ( 16.39241035757632758, -288.2596624369529650, -220.0631055782272369 ) ) ;
#54255=CARTESIAN_POINT ( 'NONE',  ( 24.38005006197849767, -288.8969061526918836, -309.6425039094027056 ) ) ;
#54256=CARTESIAN_POINT ( 'NONE',  ( -4.070783131847124814, -294.4685365476391894, -202.7343734838937337 ) ) ;
#54257=CARTESIAN_POINT ( 'NONE',  ( -31.58484446399026524, -275.0599930413331435, -345.7531370534237567 ) ) ;
#54258=CARTESIAN_POINT ( 'NONE',  ( -114.1899909918911504, -278.9414962150229371, -265.8795465218101413 ) ) ;
#54259=CARTESIAN_POINT ( 'NONE',  ( -68.99714594278383117, -289.7190220462043726, -201.7376668321577426 ) ) ;
#54260=CARTESIAN_POINT ( 'NONE',  ( -114.3778064568944473, -278.5724984469516698, -268.7342460199392349 ) ) ;
#54261=CARTESIAN_POINT ( 'NONE',  ( -68.76235899478038505, -299.6170060965190487, -202.6375507934338600 ) ) ;
#54263=CARTESIAN_POINT ( 'NONE',  ( -111.4792264354816496, -282.4020810444002905, -282.0364618641495440 ) ) ;
#54265=CARTESIAN_POINT ( 'NONE',  ( -98.68261331631168787, -276.1197464466183078, -312.1720956079731764 ) ) ;
#54266=CARTESIAN_POINT ( 'NONE',  ( 26.17159961013963709, -279.0146858647894419, -230.3756277867683480 ) ) ;
#54268=CARTESIAN_POINT ( 'NONE',  ( -17.55649340310105444, -275.2812735462158003, -344.0581555474273614 ) ) ;
#54269=CARTESIAN_POINT ( 'NONE',  ( -67.56199773301453604, -296.9760875402213856, -337.5868661549849321 ) ) ;
#54270=CARTESIAN_POINT ( 'NONE',  ( 24.84853269909145723, -281.0701806179488926, -315.2595392251381554 ) ) ;
#54271=CARTESIAN_POINT ( 'NONE',  ( -92.93080483620325083, -298.1701144406042090, -222.6631096285022693 ) ) ;
#54272=CARTESIAN_POINT ( 'NONE',  ( -113.8724468745746350, -297.8407426462014769, -272.4729998593145410 ) ) ;
#54273=CARTESIAN_POINT ( 'NONE',  ( -56.86318510286623962, -273.4602324978485512, -199.9450507135116482 ) ) ;
#54274=CARTESIAN_POINT ( 'NONE',  ( 16.28830337206679602, -294.8132240839003657, -217.8575379677758121 ) ) ;
#54275=CARTESIAN_POINT ( 'NONE',  ( 1.519845867310069432, -286.7232157719415113, -203.8718733310966513 ) ) ;
#54276=CARTESIAN_POINT ( 'NONE',  ( 11.88383322424419042, -274.5161321889597730, -327.9558429501450405 ) ) ;
#54277=CARTESIAN_POINT ( 'NONE',  ( -40.34088398147816434, -288.9221676367471900, -347.3157677629409932 ) ) ;
#54278=CARTESIAN_POINT ( 'NONE',  ( 11.29925779746202075, -285.8043899257965563, -215.5438567272127557 ) ) ;
#54279=CARTESIAN_POINT ( 'NONE',  ( -98.38794543784490543, -289.1445077773954040, -226.7909839002715842 ) ) ;
#54280=ORIENTED_EDGE ( 'NONE', *, *, #37333, .F. ) ;
#54282=CARTESIAN_POINT ( 'NONE',  ( -39.96654905466119345, -288.5935412221524530, -343.4251110606689963 ) ) ;
#54284=CARTESIAN_POINT ( 'NONE',  ( -110.4577676580129122, -285.1979998434574100, -293.7895017599760195 ) ) ;
#54285=CARTESIAN_POINT ( 'NONE',  ( 38.37221553467777824, -292.7706920483784643, -283.0986210119398834 ) ) ;
#54286=CARTESIAN_POINT ( 'NONE',  ( 35.82579292587770681, -282.8820415415041793, -249.0315653850595936 ) ) ;
#54287=CARTESIAN_POINT ( 'NONE',  ( 39.12742986579735316, -282.8975608405727939, -272.7632898019847971 ) ) ;
#54288=CARTESIAN_POINT ( 'NONE',  ( -84.86338689133147284, -283.5626794147622149, -325.7749185349479148 ) ) ;
#54289=CARTESIAN_POINT ( 'NONE',  ( -15.78223258401995466, -278.7735471704858128, -342.2500475701118035 ) ) ;
#54290=CARTESIAN_POINT ( 'NONE',  ( -114.1208200687033383, -296.6333268327786641, -263.8704576249846241 ) ) ;
#54291=CARTESIAN_POINT ( 'NONE',  ( -8.794634858030523361, -275.7486761903030583, -202.5845589780735168 ) ) ;
#54292=CARTESIAN_POINT ( 'NONE',  ( -58.08844729270684581, -289.8030236876819004, -198.6033643427983861 ) ) ;
#54293=CARTESIAN_POINT ( 'NONE',  ( -108.9187350773352421, -271.5601969347183058, -254.1173938365915888 ) ) ;
#54296=CARTESIAN_POINT ( 'NONE',  ( -103.0306629604617825, -286.0030208859412824, -305.4889604292825993 ) ) ;
#54297=CARTESIAN_POINT ( 'NONE',  ( 26.26309263966161822, -295.1986084039461389, -313.2087882425091721 ) ) ;
#54298=CARTESIAN_POINT ( 'NONE',  ( -77.11146713443663714, -286.1553927568982658, -208.9638037404032502 ) ) ;
#54299=CARTESIAN_POINT ( 'NONE',  ( 28.88687997502078275, -275.1176961439708748, -309.1760041730879038 ) ) ;
#54300=CARTESIAN_POINT ( 'NONE',  ( -68.29535452788744010, -292.3075627570773918, -199.9537009809486108 ) ) ;
#54301=CARTESIAN_POINT ( 'NONE',  ( -113.1054644874674011, -282.6967792829082669, -269.9642705730184389 ) ) ;
#54302=CARTESIAN_POINT ( 'NONE',  ( -27.85590764017713283, -292.5026065360077041, -193.9152860027418797 ) ) ;
#54303=CARTESIAN_POINT ( 'NONE',  ( -88.67291715428244459, -290.1305208578724546, -322.2956310287819406 ) ) ;
#54306=CARTESIAN_POINT ( 'NONE',  ( 173.7762727166613956, 240.3961790201574331, -177.1038114315761050 ) ) ;
#54307=CARTESIAN_POINT ( 'NONE',  ( -111.6886213027323294, -286.2891139365405024, -253.1784794286780027 ) ) ;
#54308=CARTESIAN_POINT ( 'NONE',  ( -110.4542110544635705, -294.2666405000204577, -253.6410175316879361 ) ) ;
#54310=CARTESIAN_POINT ( 'NONE',  ( 19.08279215259122452, -279.8113409422058453, -223.5388233256990418 ) ) ;
#54311=CARTESIAN_POINT ( 'NONE',  ( -34.29618122368770372, -276.6815611411086024, -347.2797055033150855 ) ) ;
#54312=CARTESIAN_POINT ( 'NONE',  ( -102.4183647061939837, -281.0459011251180641, -233.4144516712925679 ) ) ;
#54313=CARTESIAN_POINT ( 'NONE',  ( 169.6295731601628347, 230.2267480612287329, -191.3574351880446045 ) ) ;
#54314=CARTESIAN_POINT ( 'NONE',  ( -92.02482966979169987, -282.3891808533316521, -323.7311623510848904 ) ) ;
#54315=CARTESIAN_POINT ( 'NONE',  ( -109.6150329445279112, -282.8132396817231324, -251.6953158487823430 ) ) ;
#54316=CARTESIAN_POINT ( 'NONE',  ( -104.5247966912737070, -274.8730284687417225, -235.2228534304302343 ) ) ;
#54317=CARTESIAN_POINT ( 'NONE',  ( -35.64290255593734713, -295.5226499768471058, -343.4154107262830280 ) ) ;
#54319=CARTESIAN_POINT ( 'NONE',  ( 22.21410783344179052, -291.6383679442908488, -227.2775563091246340 ) ) ;
#54320=CARTESIAN_POINT ( 'NONE',  ( -41.37079839258058911, -277.7530114182702050, -347.1667514060834492 ) ) ;
#54321=CARTESIAN_POINT ( 'NONE',  ( 34.84165639972377448, -275.4074030803654409, -259.3883461098668022 ) ) ;
#54322=CARTESIAN_POINT ( 'NONE',  ( 13.76875386746906216, -273.6689094343150828, -213.1130992726049556 ) ) ;
#54324=CARTESIAN_POINT ( 'NONE',  ( -103.9237073279815462, -271.0102920859906703, -235.7266728840971552 ) ) ;
#54325=CARTESIAN_POINT ( 'NONE',  ( 25.24255633223820894, -295.5618059826121566, -314.2224950278564393 ) ) ;
#54330=CARTESIAN_POINT ( 'NONE',  ( -18.64357965821731611, -283.8854354482718350, -341.2982047164005053 ) ) ;
#54331=CARTESIAN_POINT ( 'NONE',  ( 26.98145658973689365, -282.7743815291684655, -229.8088093915696390 ) ) ;
#54332=CARTESIAN_POINT ( 'NONE',  ( -107.8616777658547363, -283.6461190332594811, -289.6652264153267424 ) ) ;
#54333=CARTESIAN_POINT ( 'NONE',  ( -40.56083621764730651, -275.4931399487513772, -344.1034791841074139 ) ) ;
#54334=CARTESIAN_POINT ( 'NONE',  ( 23.61230036274744393, -283.9933043814972962, -312.7341672628170386 ) ) ;
#54335=CARTESIAN_POINT ( 'NONE',  ( -106.9252270675567900, -276.7104583770554314, -294.7820326538454765 ) ) ;
#54336=CARTESIAN_POINT ( 'NONE',  ( 35.14524295344944704, -276.4869002304594119, -259.3282821274389676 ) ) ;
#54339=CARTESIAN_POINT ( 'NONE',  ( -50.92115537272334791, -280.6856905532321775, -194.7320414623887643 ) ) ;
#54341=DIRECTION ( 'NONE',  ( 0.000000000000000000, 0.000000000000000000, 1.000000000000000000 ) ) ;
#54342=CARTESIAN_POINT ( 'NONE',  ( -112.5955659863347478, -286.5242158929484617, -261.5769758555161957 ) ) ;
#54343=CARTESIAN_POINT ( 'NONE',  ( -35.65712385050216682, -294.2276797161182458, -343.5157222871457634 ) ) ;
#54345=CARTESIAN_POINT ( 'NONE',  ( -105.0701169924137304, -289.4292898113963020, -306.7777945929239536 ) ) ;
#54346=CARTESIAN_POINT ( 'NONE',  ( 36.64189138387394706, -285.8371288707806457, -273.8293602605959336 ) ) ;
#54347=CARTESIAN_POINT ( 'NONE',  ( 34.28801370882838739, -285.9054185147584235, -253.4377257516967177 ) ) ;
#54348=CARTESIAN_POINT ( 'NONE',  ( -111.3202212809849243, -288.7454923422922661, -273.9358544989065649 ) ) ;
#54349=CARTESIAN_POINT ( 'NONE',  ( -65.45366311071562393, -284.6331225364976945, -338.1748484081325614 ) ) ;
#54350=CARTESIAN_POINT ( 'NONE',  ( 34.14833287875688939, -273.8446070350688046, -293.0365635037624656 ) ) ;
#54351=CARTESIAN_POINT ( 'NONE',  ( 38.77967236081282465, -285.8954683745651550, -265.8859058378374698 ) ) ;
#54352=CARTESIAN_POINT ( 'NONE',  ( -79.52182682176520245, -299.4829905177365390, -208.2838452961748601 ) ) ;
#54353=CARTESIAN_POINT ( 'NONE',  ( 19.17716402239479123, -286.2390077313106644, -319.9349797677945162 ) ) ;
#54355=CARTESIAN_POINT ( 'NONE',  ( 31.28661004284614222, -282.1517877656277733, -244.6508050043901505 ) ) ;
#54356=CARTESIAN_POINT ( 'NONE',  ( -37.47221339726154099, -291.0539023684440849, -345.5404367147966695 ) ) ;
#54358=CARTESIAN_POINT ( 'NONE',  ( -97.11994273655210463, -297.8436128276508157, -316.5766555478507485 ) ) ;
#54359=CARTESIAN_POINT ( 'NONE',  ( -71.83954586158834843, -277.5960702478371331, -203.7516071013835699 ) ) ;
#54360=CARTESIAN_POINT ( 'NONE',  ( -27.85885903047549661, -291.3666758245070696, -194.0564273165381906 ) ) ;
#54361=CARTESIAN_POINT ( 'NONE',  ( -108.9462434943731921, -295.1858563333981920, -252.4424377755413786 ) ) ;
#54362=CARTESIAN_POINT ( 'NONE',  ( 20.91705214173948235, -279.6104835098763033, -225.5393043626210101 ) ) ;
#54363=CARTESIAN_POINT ( 'NONE',  ( 18.37939749841876846, -272.9396768566480205, -220.9240605947728113 ) ) ;
#54364=CARTESIAN_POINT ( 'NONE',  ( 19.22331240470157709, -295.5283291280866251, -317.2827850093944448 ) ) ;
#54365=CARTESIAN_POINT ( 'NONE',  ( 39.58706461736020543, -296.0519495502701943, -270.3284710469133074 ) ) ;
#54366=CARTESIAN_POINT ( 'NONE',  ( -107.5290224979771807, -271.5161465874575697, -240.0223143437607973 ) ) ;
#54367=CARTESIAN_POINT ( 'NONE',  ( -3.697879230575534582, -292.8542783376716443, -338.5082465673480101 ) ) ;
#54368=CARTESIAN_POINT ( 'NONE',  ( -63.02323098353827646, -293.1363140260699538, -201.3985637232659371 ) ) ;
#54370=CARTESIAN_POINT ( 'NONE',  ( 35.36859930742924263, -294.4676364044116781, -278.9192985079345135 ) ) ;
#54372=CARTESIAN_POINT ( 'NONE',  ( -95.91029375534257895, -281.9222890578718648, -317.7958171708838790 ) ) ;
#54373=CARTESIAN_POINT ( 'NONE',  ( -38.34229317417686644, -295.0650408441347849, -343.3542602190476032 ) ) ;
#54374=CARTESIAN_POINT ( 'NONE',  ( 37.86552806408568017, -281.7595048671323639, -286.9408716284606271 ) ) ;
#54375=CARTESIAN_POINT ( 'NONE',  ( -21.73442281157464606, -282.5240722037501087, -345.7412027941464316 ) ) ;
#54376=CARTESIAN_POINT ( 'NONE',  ( 13.38017965774569440, -286.3408371401578165, -325.4525892238079905 ) ) ;
#54378=CARTESIAN_POINT ( 'NONE',  ( 35.93934562868398785, -279.7622950456687931, -249.0399271567522703 ) ) ;
#54379=CARTESIAN_POINT ( 'NONE',  ( 33.75059532463390610, -286.8407465208177314, -299.2666853064187080 ) ) ;
#54381=CARTESIAN_POINT ( 'NONE',  ( -31.51912926246497193, -296.5776929383341098, -343.9817338471044081 ) ) ;
#54382=CARTESIAN_POINT ( 'NONE',  ( 20.38709532053276163, -277.6592569973349782, -320.4408157471359573 ) ) ;
#54383=CARTESIAN_POINT ( 'NONE',  ( -79.06347333526062471, -279.1385904977764199, -210.4329849635005871 ) ) ;
#54384=CARTESIAN_POINT ( 'NONE',  ( -33.54148808690165851, -292.2654278876781859, -193.4549518256146712 ) ) ;
#54385=CARTESIAN_POINT ( 'NONE',  ( -30.37251406328121561, -281.0444921009496966, -345.5990382302692865 ) ) ;
#54386=CARTESIAN_POINT ( 'NONE',  ( -91.86213878092823393, -279.8295787473639962, -321.9382570641489565 ) ) ;
#54388=CARTESIAN_POINT ( 'NONE',  ( 32.56785208163888257, -292.8991055851751071, -292.1799850036206863 ) ) ;
#54389=CARTESIAN_POINT ( 'NONE',  ( -108.8970957867788769, -294.8438361496554876, -247.7208165099362134 ) ) ;
#54392=CARTESIAN_POINT ( 'NONE',  ( 14.35539498686518911, -293.8090642734588300, -322.0597462178400292 ) ) ;
#54395=CARTESIAN_POINT ( 'NONE',  ( -53.35057174420112602, -286.7666405000204577, -340.3538533559490702 ) ) ;
#54396=CARTESIAN_POINT ( 'NONE',  ( -35.46697519860013159, -297.1338385394712986, -193.5967014325774755 ) ) ;
#54397=CARTESIAN_POINT ( 'NONE',  ( 36.92993136920981811, -279.8819839520191408, -285.3287576796730036 ) ) ;
#54398=CARTESIAN_POINT ( 'NONE',  ( -82.99511457280848958, -286.7575166729280340, -208.9023401924321774 ) ) ;
#54399=CARTESIAN_POINT ( 'NONE',  ( -15.85367591066476756, -288.5997766288515436, -340.1797280768398650 ) ) ;
#54400=CARTESIAN_POINT ( 'NONE',  ( -102.4606320305192497, -279.6067401586857386, -304.8608637575646867 ) ) ;
#54401=CARTESIAN_POINT ( 'NONE',  ( -101.4224178539420365, -274.6496410711240515, -233.6509016872105917 ) ) ;
#54402=CARTESIAN_POINT ( 'NONE',  ( -107.6028111018489568, -277.6265711124902964, -249.1359727553659411 ) ) ;
#54404=CARTESIAN_POINT ( 'NONE',  ( -106.8423102469622279, -272.8103974973882941, -237.2149990907893482 ) ) ;
#54405=CARTESIAN_POINT ( 'NONE',  ( -111.8089503080287699, -292.4970529479311381, -268.4486911278731895 ) ) ;
#54406=CARTESIAN_POINT ( 'NONE',  ( 36.30409391824681364, -294.9041970755569650, -250.7471522297435911 ) ) ;
#54409=CARTESIAN_POINT ( 'NONE',  ( -74.76096257510376120, -290.2159045468530394, -333.1746417710294850 ) ) ;
#54412=CARTESIAN_POINT ( 'NONE',  ( -55.86352057578385200, -289.9558712258774449, -196.8410936523945338 ) ) ;
#54413=CARTESIAN_POINT ( 'NONE',  ( -46.13167228009177734, -298.2768267962699156, -193.8857580223321122 ) ) ;
#54414=CARTESIAN_POINT ( 'NONE',  ( -109.1636984043707059, -296.0441523720942314, -283.6094826944226952 ) ) ;
#54417=CARTESIAN_POINT ( 'NONE',  ( -86.91913933143823101, -291.2473279656440468, -328.4372740890796081 ) ) ;
#54418=CARTESIAN_POINT ( 'NONE',  ( -88.52914483777347243, -287.9090924074130839, -206.2264541496106460 ) ) ;
#54419=CARTESIAN_POINT ( 'NONE',  ( -109.1439830577171222, -286.2796852825553060, -291.4890497068415129 ) ) ;
#54420=CARTESIAN_POINT ( 'NONE',  ( -57.32733597892497812, -271.7936214747699069, -198.1918778335514446 ) ) ;
#54421=CARTESIAN_POINT ( 'NONE',  ( -95.75765809036667520, -275.1107692989325528, -224.2212213932562008 ) ) ;
#54422=CARTESIAN_POINT ( 'NONE',  ( 24.55187252496682859, -291.0687826493541479, -229.0029281984327838 ) ) ;
#54423=CARTESIAN_POINT ( 'NONE',  ( -112.5372564876072943, -280.2894757188504400, -280.0454992716609581 ) ) ;
#54425=CARTESIAN_POINT ( 'NONE',  ( 11.97935973491609651, -281.6930745809910945, -324.3178202716776468 ) ) ;
#54426=CARTESIAN_POINT ( 'NONE',  ( 33.90222610867350994, -276.9950082340621407, -298.8908951164094674 ) ) ;
#54427=CARTESIAN_POINT ( 'NONE',  ( 19.84255179703608363, -279.6523162412574948, -219.3711039045785185 ) ) ;
#54428=CARTESIAN_POINT ( 'NONE',  ( 178.0273201536632257, 252.5904144576495014, -164.6784170649348766 ) ) ;
#54429=CARTESIAN_POINT ( 'NONE',  ( 28.29512180978152358, -275.9710213066081792, -230.4521396472545405 ) ) ;
#54430=CARTESIAN_POINT ( 'NONE',  ( -85.38682883930376022, -274.9218266514497486, -211.0789675660428770 ) ) ;
#54431=EDGE_CURVE ( 'NONE', #64642, #47196, #13662, .T. ) ;
#54432=CARTESIAN_POINT ( 'NONE',  ( 39.58706461736021254, -296.0519495502702512, -270.3284710469133074 ) ) ;
#54434=DIRECTION ( 'NONE',  ( 1.000000000000000000, 0.000000000000000000, 0.000000000000000000 ) ) ;
#54435=CARTESIAN_POINT ( 'NONE',  ( -101.9089116334536840, -291.1591002118069014, -305.1861577145047022 ) ) ;
#54436=CARTESIAN_POINT ( 'NONE',  ( 37.78033276558921472, -289.1663350957921921, -258.8442455734470968 ) ) ;
#54437=CARTESIAN_POINT ( 'NONE',  ( -108.5248306026289953, -290.1206457123464020, -253.6676062462082655 ) ) ;
#54438=CARTESIAN_POINT ( 'NONE',  ( -37.97564309066880384, -285.5520647543452810, -193.4252679523327458 ) ) ;
#54440=CARTESIAN_POINT ( 'NONE',  ( 36.31959538717714508, -279.8930026078488140, -265.8385129279841408 ) ) ;
#54441=CARTESIAN_POINT ( 'NONE',  ( 36.78451083480545947, -289.3492861351845136, -265.4823095329641092 ) ) ;
#54442=CARTESIAN_POINT ( 'NONE',  ( -59.17181237061875265, -281.8195986827554975, -340.8005201523357641 ) ) ;
#54443=CARTESIAN_POINT ( 'NONE',  ( -102.6014456462129090, -280.3252169892650159, -236.4507699486624404 ) ) ;
#54444=CARTESIAN_POINT ( 'NONE',  ( -36.45914523175086686, -277.5331807899437990, -343.4298037444884812 ) ) ;
#54445=CARTESIAN_POINT ( 'NONE',  ( -104.8135185261363347, -288.8757164180376549, -306.6318009042486210 ) ) ;
#54446=CARTESIAN_POINT ( 'NONE',  ( -65.82702165380304393, -286.4917062697573442, -198.9835192167049058 ) ) ;
#54447=CARTESIAN_POINT ( 'NONE',  ( 26.30293161275466218, -287.4737865011771873, -227.1069514626154557 ) ) ;
#54448=CARTESIAN_POINT ( 'NONE',  ( -101.7702292538398723, -284.2498290624740775, -304.7901875457919232 ) ) ;
#54451=CARTESIAN_POINT ( 'NONE',  ( -106.5925894201528337, -292.0124647025996296, -301.2247297463323434 ) ) ;
#54452=CARTESIAN_POINT ( 'NONE',  ( 21.89410770461774192, -292.8913413935417225, -318.8008619264896311 ) ) ;
#54453=CARTESIAN_POINT ( 'NONE',  ( -16.56246095852513633, -273.3859277990574697, -200.0826597055976777 ) ) ;
#54455=CARTESIAN_POINT ( 'NONE',  ( -36.28418253748976952, -294.3878474433843166, -347.2650000588765238 ) ) ;
#54457=CARTESIAN_POINT ( 'NONE',  ( -64.30745914991398138, -290.1736620626411423, -201.7649851151369944 ) ) ;
#54458=CARTESIAN_POINT ( 'NONE',  ( -38.37866671362825599, -293.3051844867461568, -344.3671901427292141 ) ) ;
#54459=CARTESIAN_POINT ( 'NONE',  ( -110.7024287695699343, -291.7102320630364716, -273.9435572138833095 ) ) ;
#54461=CARTESIAN_POINT ( 'NONE',  ( 37.41094597726377913, -291.6590403484484000, -278.7169887414202094 ) ) ;
#54463=CARTESIAN_POINT ( 'NONE',  ( 32.07424567187151609, -295.1803830892341693, -241.8280986703765905 ) ) ;
#54464=CARTESIAN_POINT ( 'NONE',  ( -10.62713326415700088, -289.6363320438476308, -338.6045173212468171 ) ) ;
#54465=CARTESIAN_POINT ( 'NONE',  ( -41.13573637961724216, -275.9846464159625725, -195.0503442723845637 ) ) ;
#54466=CARTESIAN_POINT ( 'NONE',  ( -20.22981193432151770, -275.6320915079082852, -345.0827602815496107 ) ) ;
#54467=CARTESIAN_POINT ( 'NONE',  ( -105.1063686738797287, -296.2196952535776973, -234.0252365674405439 ) ) ;
#54468=CARTESIAN_POINT ( 'NONE',  ( 33.05518132158856304, -274.0910608151258998, -293.2139754746388007 ) ) ;
#54469=CARTESIAN_POINT ( 'NONE',  ( -8.670559923868280450, -278.5101322999274771, -201.6641026272448300 ) ) ;
#54470=CARTESIAN_POINT ( 'NONE',  ( 0.8058092377127793471, -275.7784532944953639, -207.6562694148844912 ) ) ;
#54471=CARTESIAN_POINT ( 'NONE',  ( -108.9915789874954868, -276.6192475293553343, -296.4527298158090503 ) ) ;
#54474=CARTESIAN_POINT ( 'NONE',  ( -57.96005601167394161, -298.5817182397422584, -200.1650701792778762 ) ) ;
#54476=CARTESIAN_POINT ( 'NONE',  ( -72.43082167610883459, -287.5342421131651918, -337.0625941492019138 ) ) ;
#54477=CARTESIAN_POINT ( 'NONE',  ( -59.47362139256243552, -273.5909040891444306, -200.7439959945896817 ) ) ;
#54478=CARTESIAN_POINT ( 'NONE',  ( 27.44479758920837043, -288.0991780399880895, -312.0732463744585630 ) ) ;
#54479=CARTESIAN_POINT ( 'NONE',  ( -78.12880367227818112, -289.2509574530789109, -335.7084934262737193 ) ) ;
#54480=CARTESIAN_POINT ( 'NONE',  ( -92.81001138722074018, -275.2592177801483331, -219.6144523142734215 ) ) ;
#54481=CARTESIAN_POINT ( 'NONE',  ( -94.49876758437574154, -293.8822009918490608, -318.6831317049116024 ) ) ;
#54482=CARTESIAN_POINT ( 'NONE',  ( 38.70998244283266132, -280.8867824533791122, -281.3292718194990698 ) ) ;
#54484=CARTESIAN_POINT ( 'NONE',  ( -109.5562099720875864, -276.2909298093215966, -290.6578354480366215 ) ) ;
#54486=CARTESIAN_POINT ( 'NONE',  ( -98.62265046143760117, -289.9053918361510682, -229.8735844226685856 ) ) ;
#54489=CARTESIAN_POINT ( 'NONE',  ( -36.14946984881695613, -290.0669091128396531, -195.3577723839173359 ) ) ;
#54490=CARTESIAN_POINT ( 'NONE',  ( -13.86269615307618253, -275.8825680621578158, -200.5080999809406137 ) ) ;
#54491=CARTESIAN_POINT ( 'NONE',  ( 17.41678598021902857, -283.7143677768175962, -323.7294654170661374 ) ) ;
#54492=CARTESIAN_POINT ( 'NONE',  ( -112.9007917339342129, -270.6681687357510100, -267.5228849028574700 ) ) ;
#54493=CARTESIAN_POINT ( 'NONE',  ( -101.7712277623508186, -284.0831758459888761, -304.7883187367004894 ) ) ;
#54494=CARTESIAN_POINT ( 'NONE',  ( -1.450986670879202078, -275.9632052979118271, -206.1031571055587790 ) ) ;
#54495=CARTESIAN_POINT ( 'NONE',  ( -40.79276897210233699, -274.8106091891630740, -197.2312705246400526 ) ) ;
#54496=CARTESIAN_POINT ( 'NONE',  ( 24.30143081559814533, -284.1319473691979738, -313.1051977790644401 ) ) ;
#54497=CARTESIAN_POINT ( 'NONE',  ( -110.1914158896640572, -271.5801148496640849, -262.1669135185482560 ) ) ;
#54500=CARTESIAN_POINT ( 'NONE',  ( -32.01462874864632369, -294.8200442288518843, -347.1898808266892615 ) ) ;
#54501=CARTESIAN_POINT ( 'NONE',  ( -111.1202223974959509, -286.3814913097627368, -282.0311711577576830 ) ) ;
#54503=CARTESIAN_POINT ( 'NONE',  ( -55.56934967048407970, -271.3380690714491266, -190.3538533559490702 ) ) ;
#54504=CARTESIAN_POINT ( 'NONE',  ( -48.48070493199901421, -276.3875361728109965, -346.4417467637877053 ) ) ;
#54505=CARTESIAN_POINT ( 'NONE',  ( -111.1522676921088504, -288.7120185491118605, -289.3458983780992071 ) ) ;
#54506=CARTESIAN_POINT ( 'NONE',  ( -36.16321116965146132, -284.5572351284840806, -344.0450301899877559 ) ) ;
#54507=CARTESIAN_POINT ( 'NONE',  ( -105.1914927648264921, -279.9186217476672596, -300.0593613551778844 ) ) ;
#54508=CARTESIAN_POINT ( 'NONE',  ( -75.82577573433958662, -286.9745526073546671, -204.2881945408871331 ) ) ;
#54509=CARTESIAN_POINT ( 'NONE',  ( 25.34042337187527494, -282.9954566652615995, -229.0855679903297073 ) ) ;
#54510=CARTESIAN_POINT ( 'NONE',  ( 18.08812233331095243, -274.9863233189198013, -216.8380205676778871 ) ) ;
#54511=CARTESIAN_POINT ( 'NONE',  ( -51.31470074704450468, -277.0594005603667256, -346.0826820062148386 ) ) ;
#54512=CARTESIAN_POINT ( 'NONE',  ( -12.50519009885741539, -296.6469471360258012, -340.5899450461357674 ) ) ;
#54513=DIRECTION ( 'NONE',  ( 0.000000000000000000, -1.000000000000000000, 0.000000000000000000 ) ) ;
#54515=CIRCLE ( 'NONE', #78745, 0.5000000000000004441 ) ;
#54516=CARTESIAN_POINT ( 'NONE',  ( -43.17070068259021554, -296.1190206143008368, -194.7685192277762951 ) ) ;
#54517=CARTESIAN_POINT ( 'NONE',  ( -101.9142347688244428, -277.5945949126103187, -304.5426365495230243 ) ) ;
#54518=CARTESIAN_POINT ( 'NONE',  ( -75.63752434942367131, -298.6336778810543251, -203.8552832132004937 ) ) ;
#54519=AXIS2_PLACEMENT_3D ( 'NONE', #39930, #18643, #32851 ) ;
#54520=CARTESIAN_POINT ( 'NONE',  ( -35.93639475293624486, -287.8301596497616401, -196.3611238416436038 ) ) ;
#54521=CARTESIAN_POINT ( 'NONE',  ( -97.71393025181423297, -297.4436454701123012, -317.0291111367592407 ) ) ;
#54522=CARTESIAN_POINT ( 'NONE',  ( -27.78209149001932943, -296.1385359950452880, -346.4182321894500092 ) ) ;
#54523=CARTESIAN_POINT ( 'NONE',  ( -111.7995127460078066, -292.6486687502030577, -262.8736240630379939 ) ) ;
#54524=CARTESIAN_POINT ( 'NONE',  ( -35.59509969697922571, -278.0739276924878709, -195.5354518844400218 ) ) ;
#54525=CARTESIAN_POINT ( 'NONE',  ( -96.77595910661851519, -281.0899245823202364, -225.5193859641550773 ) ) ;
#54526=CARTESIAN_POINT ( 'NONE',  ( -108.7630797693000204, -270.8553139343745215, -248.4855661378616105 ) ) ;
#54527=CARTESIAN_POINT ( 'NONE',  ( -5.945400681139366483, -284.5042479926262899, -339.3145650658788668 ) ) ;
#54528=CARTESIAN_POINT ( 'NONE',  ( 34.01435421217547628, -286.2509634147783686, -253.4979098905831165 ) ) ;
#54529=CARTESIAN_POINT ( 'NONE',  ( -76.26301331016580320, -209.3917711165195499, -356.8240937122167225 ) ) ;
#54531=CARTESIAN_POINT ( 'NONE',  ( -37.27659351975641755, -285.7196708280350776, -197.3275608611384371 ) ) ;
#54533=CARTESIAN_POINT ( 'NONE',  ( -61.12270646156451903, -284.4333553756609945, -343.3271794767043730 ) ) ;
#54534=CARTESIAN_POINT ( 'NONE',  ( -21.93370400848765911, -274.5883638998539027, -198.9840828644169903 ) ) ;
#54535=CARTESIAN_POINT ( 'NONE',  ( 26.81363734757852768, -285.7943436032209661, -228.5030077566260047 ) ) ;
#54536=CARTESIAN_POINT ( 'NONE',  ( -7.639133801106644306, -281.3733196298504708, -199.5614249559657765 ) ) ;
#54538=CARTESIAN_POINT ( 'NONE',  ( -113.6908671728898241, -280.0564305816117212, -271.6164854738045733 ) ) ;
#54539=CARTESIAN_POINT ( 'NONE',  ( 37.52879818320447214, -282.1099233519890959, -288.3101705966004715 ) ) ;
#54540=CARTESIAN_POINT ( 'NONE',  ( -92.08974858914540107, -287.4094976428775112, -313.9805196606274080 ) ) ;
#54541=CARTESIAN_POINT ( 'NONE',  ( -77.26738670498112072, -208.9735159622803167, -357.2724075973424647 ) ) ;
#54543=CARTESIAN_POINT ( 'NONE',  ( -60.05576592190065810, -275.7573956509355071, -199.0039877813583189 ) ) ;
#54544=CARTESIAN_POINT ( 'NONE',  ( -13.59065996674749499, -91.27732092402939656, -359.7254001870301181 ) ) ;
#54545=CARTESIAN_POINT ( 'NONE',  ( 33.54640980252191440, -279.2668085063594390, -246.8159353152754534 ) ) ;
#54546=CARTESIAN_POINT ( 'NONE',  ( 38.59504438108795910, -295.3471959517924006, -273.1151776711053003 ) ) ;
#54547=CARTESIAN_POINT ( 'NONE',  ( -106.9689028769844157, -295.6038704980115313, -292.7948782161178656 ) ) ;
#54548=CARTESIAN_POINT ( 'NONE',  ( -53.37037148213816806, -291.3596647568022604, -195.0563583117382791 ) ) ;
#54550=CARTESIAN_POINT ( 'NONE',  ( -96.95920022519082693, -294.4813783000894887, -318.1768096104395909 ) ) ;
#54551=CARTESIAN_POINT ( 'NONE',  ( 36.45495667822554964, -285.9611860073666776, -271.0638677363292004 ) ) ;
#54552=CARTESIAN_POINT ( 'NONE',  ( 15.74248330177986688, -294.6735020686085136, -218.3940209165518240 ) ) ;
#54553=CARTESIAN_POINT ( 'NONE',  ( -110.8837751754803804, -285.8598831551734065, -270.9297172159879210 ) ) ;
#54554=VERTEX_POINT ( 'NONE', #67932 ) ;
#54555=CARTESIAN_POINT ( 'NONE',  ( 1.570458592538932496, -293.4998677468823871, -204.1289002139018578 ) ) ;
#54556=CARTESIAN_POINT ( 'NONE',  ( -38.88009359107142870, -283.5642802192047043, -343.4189600977773011 ) ) ;
#54557=CARTESIAN_POINT ( 'NONE',  ( -55.98855466317340301, -294.0820598187446535, -344.6598631497901124 ) ) ;
#54558=CARTESIAN_POINT ( 'NONE',  ( -100.5419534657935685, -290.7766098925367828, -314.0633696249525997 ) ) ;
#54559=CARTESIAN_POINT ( 'NONE',  ( -98.30335177756714415, -291.6715516409488487, -223.4014985039431451 ) ) ;
#54560=CARTESIAN_POINT ( 'NONE',  ( -66.32707632853670532, -289.6090687285297918, -337.4139987518576618 ) ) ;
#54563=CARTESIAN_POINT ( 'NONE',  ( -110.7656478456406290, -298.1743065953174892, -289.1011075472248990 ) ) ;
#54564=CARTESIAN_POINT ( 'NONE',  ( -113.9440573844913445, -271.3831319911222977, -267.4931300989931060 ) ) ;
#54565=CARTESIAN_POINT ( 'NONE',  ( -35.64537022646563003, -279.1326649175781540, -197.1330287555149710 ) ) ;
#54567=CARTESIAN_POINT ( 'NONE',  ( -3.847224832576078946, -273.9898579218531722, -201.0815712984729942 ) ) ;
#54568=CARTESIAN_POINT ( 'NONE',  ( -65.82296942945141893, -296.1525263929442531, -202.3940299736871395 ) ) ;
#54569=CARTESIAN_POINT ( 'NONE',  ( -43.28271581739778640, -278.9883950154219292, -344.3582112572414076 ) ) ;
#54570=CARTESIAN_POINT ( 'NONE',  ( 3.631105760235500135, -272.7489587030858047, -208.3957567974503320 ) ) ;
#54571=CARTESIAN_POINT ( 'NONE',  ( -96.72066180132647162, -297.1564465682660625, -313.5249958836847668 ) ) ;
#54572=CARTESIAN_POINT ( 'NONE',  ( -50.02083663284555115, -298.9662226655478321, -198.1567859083824032 ) ) ;
#54573=CARTESIAN_POINT ( 'NONE',  ( 128.9960186029002500, -299.5541904835127980, -195.3611179825600175 ) ) ;
#54574=CARTESIAN_POINT ( 'NONE',  ( -113.5654007414033373, -298.1256511623388405, -272.4682174214288466 ) ) ;
#54575=CARTESIAN_POINT ( 'NONE',  ( -91.96220046314745389, -271.2974590167983706, -218.4288306385668932 ) ) ;
#54576=CARTESIAN_POINT ( 'NONE',  ( 19.41969872385966411, -293.5525080588010383, -224.2757582449652034 ) ) ;
#54577=CARTESIAN_POINT ( 'NONE',  ( -82.07293585013043469, -290.0036531682835630, -211.8629982991163274 ) ) ;
#54578=CARTESIAN_POINT ( 'NONE',  ( 28.56507200901022259, -300.8773574837633760, -195.3386412410832236 ) ) ;
#54579=CARTESIAN_POINT ( 'NONE',  ( 28.44667063823031938, -275.5221888306387541, -230.3667112173299643 ) ) ;
#54580=CARTESIAN_POINT ( 'NONE',  ( -110.3417791297764268, -272.7547376145998896, -267.6393759378285608 ) ) ;
#54581=CARTESIAN_POINT ( 'NONE',  ( -30.34203013114005287, -284.9439093263915197, -345.3905217009919966 ) ) ;
#54582=CARTESIAN_POINT ( 'NONE',  ( -4.391495585576476124, -281.3117872631973455, -339.4231938077035124 ) ) ;
#54583=CARTESIAN_POINT ( 'NONE',  ( -74.05549271712872894, -276.8753756295446351, -337.9439202656499788 ) ) ;
#54585=CARTESIAN_POINT ( 'NONE',  ( -104.7423399430342101, -284.1319670707478622, -241.7747436285103504 ) ) ;
#54586=CARTESIAN_POINT ( 'NONE',  ( 36.85399159966266325, -279.7073047883271215, -282.4841003916467344 ) ) ;
#54588=CARTESIAN_POINT ( 'NONE',  ( 10.02960774911761277, -274.9588272284195227, -326.6757173817206876 ) ) ;
#54589=CARTESIAN_POINT ( 'NONE',  ( -93.88263849894434543, -279.8681280282063994, -319.6562693588560364 ) ) ;
#54591=CARTESIAN_POINT ( 'NONE',  ( -23.56584007183121443, -296.4622326768405287, -194.3785059543251634 ) ) ;
#54593=CARTESIAN_POINT ( 'NONE',  ( -108.9130038549150754, -280.2545261918359643, -293.4975626544832039 ) ) ;
#54595=CARTESIAN_POINT ( 'NONE',  ( -112.8879512033866064, -286.5126017952944153, -267.1995143589419399 ) ) ;
#54598=CARTESIAN_POINT ( 'NONE',  ( 32.55958156416060234, -285.1967721939885791, -243.0395010916681997 ) ) ;
#54600=CARTESIAN_POINT ( 'NONE',  ( -69.91400815895589460, -294.2860004362561313, -336.1347848688370732 ) ) ;
#54601=CARTESIAN_POINT ( 'NONE',  ( -2.812602291530306609, -286.7306254631795923, -336.1341462130840227 ) ) ;
#54602=CARTESIAN_POINT ( 'NONE',  ( 84.09003387609358526, 83.72762891241104910, -302.5758382668069544 ) ) ;
#54603=CARTESIAN_POINT ( 'NONE',  ( -110.2490798380144383, -294.3254077210424384, -288.0083783456177002 ) ) ;
#54604=CARTESIAN_POINT ( 'NONE',  ( -93.39713546299613256, -283.7440794876658288, -218.5101955514913357 ) ) ;
#54605=CARTESIAN_POINT ( 'NONE',  ( 36.36593196416949780, -283.2004539263394349, -274.0523758527202176 ) ) ;
#54606=CARTESIAN_POINT ( 'NONE',  ( -41.53592186549863641, -281.3440171400004033, -346.2835830417213288 ) ) ;
#54607=CARTESIAN_POINT ( 'NONE',  ( -97.34890827293364168, -289.9726988779725048, -311.9539219315899459 ) ) ;
#54608=CARTESIAN_POINT ( 'NONE',  ( -85.88638354005971109, -280.7891551208682017, -215.0548016337999115 ) ) ;
#54609=CARTESIAN_POINT ( 'NONE',  ( 32.12671149447684371, -282.0490845942538840, -247.2506649447183236 ) ) ;
#54610=CARTESIAN_POINT ( 'NONE',  ( 37.34171039266468739, -289.4037437172542013, -260.3214468990019554 ) ) ;
#54612=CARTESIAN_POINT ( 'NONE',  ( -41.19277030543477736, -274.0050740280257173, -193.4052220642227269 ) ) ;
#54613=CARTESIAN_POINT ( 'NONE',  ( -102.5730536940850328, -293.0184948177988531, -233.9682917852116475 ) ) ;
#54615=CARTESIAN_POINT ( 'NONE',  ( -115.3430155898818299, -293.2662352645559167, -252.5904736702033517 ) ) ;
#54617=CARTESIAN_POINT ( 'NONE',  ( 22.88311951804342925, -274.1649601480243632, -315.3388850242654371 ) ) ;
#54619=CARTESIAN_POINT ( 'NONE',  ( -34.90089267273180695, -293.4218464418098051, -346.5220192127906671 ) ) ;
#54620=CARTESIAN_POINT ( 'NONE',  ( -92.08900282526985848, -272.5918949972167979, -221.9191370594037949 ) ) ;
#54621=CARTESIAN_POINT ( 'NONE',  ( -70.26496703914455111, -291.0142479948054870, -336.3051166776849072 ) ) ;
#54622=CARTESIAN_POINT ( 'NONE',  ( -21.14492922431972133, -284.6018066323541120, -342.6332344950658921 ) ) ;
#54623=CARTESIAN_POINT ( 'NONE',  ( -104.1040333734418226, -292.4629509315023483, -233.1939664755869330 ) ) ;
#54624=CARTESIAN_POINT ( 'NONE',  ( -30.75651725961395044, -293.4487808718054112, -194.0857768963367675 ) ) ;
#54625=CARTESIAN_POINT ( 'NONE',  ( -60.25695242213713243, -291.5800842411453004, -200.9979695402869027 ) ) ;
#54626=CARTESIAN_POINT ( 'NONE',  ( -106.4501065661208230, -286.9345089984053061, -241.0894222994657810 ) ) ;
#54627=CARTESIAN_POINT ( 'NONE',  ( -50.94171455630022649, -280.0496404243696702, -194.5716753665946044 ) ) ;
#54628=CARTESIAN_POINT ( 'NONE',  ( -99.55094671785275295, -295.2092901966221348, -227.4510513698674288 ) ) ;
#54629=CARTESIAN_POINT ( 'NONE',  ( 13.67920063654869445, -282.1939826511066371, -328.1024246120642260 ) ) ;
#54630=CARTESIAN_POINT ( 'NONE',  ( 36.93511906904098652, -277.4284133489766191, -271.5820317081910957 ) ) ;
#54631=CARTESIAN_POINT ( 'NONE',  ( -85.33152481854864391, -299.9090924074131408, -210.2361428286349110 ) ) ;
#54632=CARTESIAN_POINT ( 'NONE',  ( -41.34328506424762395, -275.2415879886764287, -346.0331711370850485 ) ) ;
#54634=CARTESIAN_POINT ( 'NONE',  ( -58.97232724401461468, -282.8472079639431058, -340.2004394190266225 ) ) ;
#54635=CARTESIAN_POINT ( 'NONE',  ( -112.0180984976857275, -279.9718339427403180, -253.2893797217364238 ) ) ;
#54636=CARTESIAN_POINT ( 'NONE',  ( 36.55464456235706905, -286.8727627748725695, -291.1975255861840992 ) ) ;
#54637=CARTESIAN_POINT ( 'NONE',  ( -34.84524596328733992, -293.8440848399874312, -196.3898956588212172 ) ) ;
#54638=CARTESIAN_POINT ( 'NONE',  ( 26.98454783646936761, -277.6943517093479272, -311.3074249825961033 ) ) ;
#54640=CARTESIAN_POINT ( 'NONE',  ( 30.80340306003076378, -276.4165085691404897, -235.5826306243239401 ) ) ;
#54641=CARTESIAN_POINT ( 'NONE',  ( -51.28296348307339514, -277.0687124877008500, -342.0175285858742882 ) ) ;
#54643=CARTESIAN_POINT ( 'NONE',  ( -98.67165023545506131, -297.9690220861425018, -313.2407827136157152 ) ) ;
#54644=CARTESIAN_POINT ( 'NONE',  ( -105.1358189119283963, -282.9708252718825179, -238.5526307209429433 ) ) ;
#54645=CARTESIAN_POINT ( 'NONE',  ( -30.69486334076684741, -291.8005915636979353, -193.6170196874747944 ) ) ;
#54646=CARTESIAN_POINT ( 'NONE',  ( -31.86373137704978831, -290.5843758170571505, -346.4159714253527795 ) ) ;
#54647=CARTESIAN_POINT ( 'NONE',  ( 32.09825129800050547, -292.1596630215785808, -246.7015338297873939 ) ) ;
#54649=CARTESIAN_POINT ( 'NONE',  ( -74.37729085691879050, -290.1442795661108676, -203.5257133468976747 ) ) ;
#54650=CARTESIAN_POINT ( 'NONE',  ( 16.75670112267849277, -292.5156325405050097, -221.2415604654017045 ) ) ;
#54652=CARTESIAN_POINT ( 'NONE',  ( -1.931177007002584656, -289.6739066750046163, -338.3874905371809518 ) ) ;
#54653=CARTESIAN_POINT ( 'NONE',  ( -102.1766101747465996, -279.3434821536083064, -236.6575792824504560 ) ) ;
#54654=CARTESIAN_POINT ( 'NONE',  ( -102.0481846402981176, -296.0142337675970339, -229.1960433260148591 ) ) ;
#54655=CARTESIAN_POINT ( 'NONE',  ( -1.025030557997025360, -287.1727521185500223, -202.5790237529462274 ) ) ;
#54656=CARTESIAN_POINT ( 'NONE',  ( 37.48486602947158275, -288.1122165336381045, -288.4924709483038328 ) ) ;
#54657=CARTESIAN_POINT ( 'NONE',  ( -109.2145940201805132, -285.0564676951663614, -257.3921248235521944 ) ) ;
#54658=CARTESIAN_POINT ( 'NONE',  ( -71.48678950958364453, -195.9896530787580389, -360.3036401658270620 ) ) ;
#54659=CARTESIAN_POINT ( 'NONE',  ( -108.2218527567996915, -260.4523294004561649, -316.5612791343883146 ) ) ;
#54660=CARTESIAN_POINT ( 'NONE',  ( 5.250456697231451919, -59.01702808322732352, -350.9678742460372405 ) ) ;
#54662=CARTESIAN_POINT ( 'NONE',  ( -5.227969495918243226, -273.6831247920401893, -204.6105902164035228 ) ) ;
#54663=CARTESIAN_POINT ( 'NONE',  ( -8.630232360692120963, -275.5876997396466663, -337.8274976556004390 ) ) ;
#54664=CARTESIAN_POINT ( 'NONE',  ( -37.60115747517003371, -297.5566405813652295, -193.4230936677248565 ) ) ;
#54665=CARTESIAN_POINT ( 'NONE',  ( 154.5266617868613253, 204.3775580378999450, -214.7585744442969542 ) ) ;
#54666=CARTESIAN_POINT ( 'NONE',  ( 19.49951877326586924, -274.9367919269741947, -321.5898398927589596 ) ) ;
#54667=CARTESIAN_POINT ( 'NONE',  ( -94.57608344790115495, -274.9681035542974428, -223.4136971311261561 ) ) ;
#54668=CARTESIAN_POINT ( 'NONE',  ( 98.65582398152450594, -300.6570902592916354, -193.5751751503145215 ) ) ;
#54670=CARTESIAN_POINT ( 'NONE',  ( -61.26925297919074609, -289.8637906923214018, -339.3934340103310205 ) ) ;
#54671=CARTESIAN_POINT ( 'NONE',  ( -70.72844725851523151, -296.2840863250205530, -339.5816944499152328 ) ) ;
#54672=CARTESIAN_POINT ( 'NONE',  ( -113.1421496568406013, -296.8757144146825340, -283.8460706129978917 ) ) ;
#54673=CARTESIAN_POINT ( 'NONE',  ( -75.65624939782556169, -295.7453008960374063, -332.5569577960851007 ) ) ;
#54675=CARTESIAN_POINT ( 'NONE',  ( -83.95839471173226798, -279.6066080095891948, -329.8935246980554439 ) ) ;
#54677=CARTESIAN_POINT ( 'NONE',  ( 39.12234881275100662, -280.9471874417193931, -261.3633933933106164 ) ) ;
#54678=CARTESIAN_POINT ( 'NONE',  ( 18.49555896795527943, -277.1650203342973668, -317.7489745004397150 ) ) ;
#54679=CARTESIAN_POINT ( 'NONE',  ( -5.686213211836077974, -278.4016907416234403, -339.4400884786396091 ) ) ;
#54680=CARTESIAN_POINT ( 'NONE',  ( -83.87101026556891270, -275.7071893048811830, -329.7016322165442830 ) ) ;
#54681=CARTESIAN_POINT ( 'NONE',  ( -64.59756155679460221, -274.1788316492083482, -202.5604116328183579 ) ) ;
#54682=CARTESIAN_POINT ( 'NONE',  ( -41.88674800110077712, -296.5684808699012933, -196.9123776421947696 ) ) ;
#54684=CARTESIAN_POINT ( 'NONE',  ( -108.4857863948629131, -278.5023390013022890, -286.7725164683772050 ) ) ;
#54685=CARTESIAN_POINT ( 'NONE',  ( -29.04739533227477821, -287.6340839070055040, -346.4702190549190277 ) ) ;
#54686=CARTESIAN_POINT ( 'NONE',  ( -84.56910444423637330, -275.4017879252262446, -212.0981543848764090 ) ) ;
#54688=CARTESIAN_POINT ( 'NONE',  ( -110.4062734849154168, -289.8104668481442445, -265.7151985562770733 ) ) ;
#54689=CARTESIAN_POINT ( 'NONE',  ( -97.09843596767852603, -283.2505527954193667, -318.7806284116109055 ) ) ;
#54690=CARTESIAN_POINT ( 'NONE',  ( 32.94590736020091271, -279.4865240379141369, -247.0126652185127796 ) ) ;
#54691=CARTESIAN_POINT ( 'NONE',  ( 15.69655556348369885, -279.3955606098330691, -219.2753789985103481 ) ) ;
#54692=CARTESIAN_POINT ( 'NONE',  ( -88.67008483207021641, -283.4048497679304432, -216.4471947362969217 ) ) ;
#54693=CARTESIAN_POINT ( 'NONE',  ( -6.530856881225692412, -288.4568769625128084, -201.9682219244134274 ) ) ;
#54694=CARTESIAN_POINT ( 'NONE',  ( -77.04950660590047562, -280.7125181827636311, -208.5719192289845694 ) ) ;
#54696=CARTESIAN_POINT ( 'NONE',  ( -52.99736190476249931, -293.8517713645351819, -196.9602246445333549 ) ) ;
#54697=CARTESIAN_POINT ( 'NONE',  ( -112.7633383177375208, -276.6695023354861291, -280.0280531230036445 ) ) ;
#54698=CARTESIAN_POINT ( 'NONE',  ( 30.37558207583533942, -276.5735138454250546, -298.0324111229830919 ) ) ;
#54699=CARTESIAN_POINT ( 'NONE',  ( -3.690198383856922781, -284.6093846445712074, -337.5885544258872528 ) ) ;
#54701=CARTESIAN_POINT ( 'NONE',  ( -110.5211717831488158, -292.2317317432538175, -289.2298020476632132 ) ) ;
#54702=CARTESIAN_POINT ( 'NONE',  ( -109.3255128253985333, -294.2787991223954123, -291.5952737804996673 ) ) ;
#54703=CARTESIAN_POINT ( 'NONE',  ( 20.17269628375615298, -286.0569673430740636, -219.3291220171019802 ) ) ;
#54704=CARTESIAN_POINT ( 'NONE',  ( -107.3235106087011985, -289.2598391952108727, -246.9306545490687483 ) ) ;
#54706=CARTESIAN_POINT ( 'NONE',  ( 35.87106203721491227, -274.1456349666021310, -263.3905188740209837 ) ) ;
#54707=CARTESIAN_POINT ( 'NONE',  ( -73.93151162947731336, -293.6832694069670993, -334.9525351786377882 ) ) ;
#54709=CARTESIAN_POINT ( 'NONE',  ( -30.73780285809773716, -290.6139422068088152, -194.2884671063692110 ) ) ;
#54710=CARTESIAN_POINT ( 'NONE',  ( -22.31665797051880062, -287.8477652845519401, -198.0543397047241569 ) ) ;
#54711=CARTESIAN_POINT ( 'NONE',  ( 13.90356462351033962, -286.5852925128036759, -326.5385220232933534 ) ) ;
#54712=CARTESIAN_POINT ( 'NONE',  ( -110.6815248929286639, -285.8982147470362634, -276.4146309748921340 ) ) ;
#54714=CARTESIAN_POINT ( 'NONE',  ( -11.97556138708707252, -287.1937924593620437, -201.7377929952737645 ) ) ;
#54715=CARTESIAN_POINT ( 'NONE',  ( 33.93896361373181492, -295.8486607460680489, -294.9644553570703351 ) ) ;
#54716=CARTESIAN_POINT ( 'NONE',  ( -67.16321444335588353, -275.5199345788036567, -339.7872764816617064 ) ) ;
#54718=CARTESIAN_POINT ( 'NONE',  ( 39.68627834990948600, -275.8955164503840933, -271.1671843719709614 ) ) ;
#54720=CARTESIAN_POINT ( 'NONE',  ( -67.72683166957153844, -289.7364111817677212, -201.1656808762559763 ) ) ;
#54721=CARTESIAN_POINT ( 'NONE',  ( -104.7935864188600590, -279.0331759875775788, -233.2229565335078973 ) ) ;
#54722=CARTESIAN_POINT ( 'NONE',  ( -110.7553187964862502, -298.3569519150567544, -283.9331817824998438 ) ) ;
#54725=CARTESIAN_POINT ( 'NONE',  ( -109.1616785944288210, -276.9361692062703355, -251.5294449828613494 ) ) ;
#54726=CARTESIAN_POINT ( 'NONE',  ( 14.35601586795831075, -280.3251422878600465, -324.6966202592768695 ) ) ;
#54728=CARTESIAN_POINT ( 'NONE',  ( 33.08122092260052227, -273.6534324041895729, -240.8422559923055246 ) ) ;
#54730=CARTESIAN_POINT ( 'NONE',  ( 33.01444932175722613, -295.3600823442710634, -292.2864455125696281 ) ) ;
#54731=CARTESIAN_POINT ( 'NONE',  ( -52.86852594743199063, -282.1668471298895611, -345.5180576599705660 ) ) ;
#54732=CARTESIAN_POINT ( 'NONE',  ( -75.77135397721518473, -296.5197479846367514, -332.7625980591599841 ) ) ;
#54733=CARTESIAN_POINT ( 'NONE',  ( -112.9051400078289760, -298.0191312508962937, -258.3003318703342757 ) ) ;
#54734=CARTESIAN_POINT ( 'NONE',  ( -71.66312347702996988, -297.4186680807770813, -205.9183559838716064 ) ) ;
#54735=CARTESIAN_POINT ( 'NONE',  ( -16.91160945744981703, -294.3160089787164111, -198.1433045205163239 ) ) ;
#54736=CARTESIAN_POINT ( 'NONE',  ( 25.85292341809120842, -288.3012346597075179, -314.4463002195279273 ) ) ;
#54737=CARTESIAN_POINT ( 'NONE',  ( 19.87168363016981232, -274.3740997330951927, -320.0489872838214183 ) ) ;
#54738=CARTESIAN_POINT ( 'NONE',  ( 7.932796896963242084, -288.2861002955175991, -332.7102519098718290 ) ) ;
#54739=CARTESIAN_POINT ( 'NONE',  ( 3.736705292930350808, -287.5433014349188170, -331.0520649069931665 ) ) ;
#54740=CARTESIAN_POINT ( 'NONE',  ( -71.24479340915372916, -289.6044789287073513, -203.4471172219620314 ) ) ;
#54743=CARTESIAN_POINT ( 'NONE',  ( -48.07621344458673462, -288.6999170863115296, -342.6808395879009481 ) ) ;
#54745=CARTESIAN_POINT ( 'NONE',  ( -108.8138128260671778, -285.8511689784494365, -242.2065480276230005 ) ) ;
#54746=CARTESIAN_POINT ( 'NONE',  ( 36.06549682462953399, -292.3280940366882419, -247.9066385060554296 ) ) ;
#54747=CARTESIAN_POINT ( 'NONE',  ( 25.60810134203713062, -282.5789186198248899, -227.3300239028076817 ) ) ;
#54749=CARTESIAN_POINT ( 'NONE',  ( -56.44978138196967876, -281.1262038345006431, -196.2242182885780721 ) ) ;
#54750=CARTESIAN_POINT ( 'NONE',  ( -6.034869767349240632, -282.4622373114829088, -336.3209247320178292 ) ) ;
#54751=CARTESIAN_POINT ( 'NONE',  ( -4.158893940830177272, -278.6149089234165785, -337.6353494535044888 ) ) ;
#54752=CARTESIAN_POINT ( 'NONE',  ( -104.6029043052289040, -296.0649866144757993, -307.9525183963800146 ) ) ;
#54753=CARTESIAN_POINT ( 'NONE',  ( -108.1231437001084288, -288.8801366316544659, -246.6580791891732645 ) ) ;
#54754=CARTESIAN_POINT ( 'NONE',  ( -66.93155183245974627, -296.5753386398526459, -203.2752804489637413 ) ) ;
#54758=CARTESIAN_POINT ( 'NONE',  ( -109.4828344749282252, -286.2347031585719037, -288.7178861071425899 ) ) ;
#54759=CARTESIAN_POINT ( 'NONE',  ( 17.35078598243592296, -295.3735180503437050, -324.1974729756229863 ) ) ;
#54760=CARTESIAN_POINT ( 'NONE',  ( -83.71893170564314346, -286.0477156260857328, -213.7883059166572082 ) ) ;
#54761=CARTESIAN_POINT ( 'NONE',  ( -6.679727891003104823, -275.7181059702332391, -340.7504931163030051 ) ) ;
#54762=CARTESIAN_POINT ( 'NONE',  ( -90.72115765071453097, -291.9708459888942684, -214.9342829792792315 ) ) ;
#54763=CARTESIAN_POINT ( 'NONE',  ( -62.76430338365177164, -283.8642871386332445, -198.9888774174734749 ) ) ;
#54764=CARTESIAN_POINT ( 'NONE',  ( 23.95581675014300416, -293.2644875331943126, -223.7737893877462909 ) ) ;
#54765=CARTESIAN_POINT ( 'NONE',  ( -68.76323214346719226, -289.8102807075879355, -336.2760238285457035 ) ) ;
#54769=CARTESIAN_POINT ( 'NONE',  ( -88.26448419966551739, -229.6996826356688359, -344.4427272830038760 ) ) ;
#54770=CARTESIAN_POINT ( 'NONE',  ( -91.92415337550016829, -285.3341001775988843, -323.6852546341170864 ) ) ;
#54771=CARTESIAN_POINT ( 'NONE',  ( -114.2704648735229114, -282.0523547857346784, -270.3284710469133074 ) ) ;
#54773=CARTESIAN_POINT ( 'NONE',  ( 35.73595927994151822, -280.5569496626930004, -276.7918812229924015 ) ) ;
#54774=CARTESIAN_POINT ( 'NONE',  ( -2.738418744867219257, -276.2740244478974887, -339.1388427879324468 ) ) ;
#54775=CARTESIAN_POINT ( 'NONE',  ( -57.63422218619935222, -281.7897016551495994, -198.3316658654249807 ) ) ;
#54776=CARTESIAN_POINT ( 'NONE',  ( -107.0711107231528842, -266.7388540463169875, -306.2465019403078372 ) ) ;
#54777=CARTESIAN_POINT ( 'NONE',  ( 36.03897685995190869, -279.8571293983528676, -249.0096524390684749 ) ) ;
#54778=CARTESIAN_POINT ( 'NONE',  ( -82.45301188824893757, -283.4527504973215173, -210.8899791761965616 ) ) ;
#54779=CARTESIAN_POINT ( 'NONE',  ( 96.93211984402050518, -301.4714976373853119, -194.3347991198949956 ) ) ;
#54780=CARTESIAN_POINT ( 'NONE',  ( -97.23022912848335864, -296.4614522508908294, -312.2102820830003225 ) ) ;
#54782=CARTESIAN_POINT ( 'NONE',  ( -30.74614965458419036, -290.8220931753748459, -197.1645183896307572 ) ) ;
#54783=CARTESIAN_POINT ( 'NONE',  ( -48.47102471743825447, -277.8415477745168687, -346.5033817274929220 ) ) ;
#54784=CARTESIAN_POINT ( 'NONE',  ( 35.64290476491508031, -275.5323758985769018, -268.8619686860586739 ) ) ;
#54785=CARTESIAN_POINT ( 'NONE',  ( 2.270159155090923253, -273.4900990414959097, -204.6923041232815024 ) ) ;
#54787=CARTESIAN_POINT ( 'NONE',  ( -11.83557922115861949, -272.3838909394409598, -199.7769930510949905 ) ) ;
#54792=CARTESIAN_POINT ( 'NONE',  ( 3.574097049783933500, -283.5674610968012530, -331.2511711115135427 ) ) ;
#54793=CARTESIAN_POINT ( 'NONE',  ( 22.61733212670093351, -283.9443848728290050, -317.0607173630778561 ) ) ;
#54794=CARTESIAN_POINT ( 'NONE',  ( -94.19609121023967191, -284.5498958438442969, -224.3905375875953041 ) ) ;
#54795=CARTESIAN_POINT ( 'NONE',  ( -74.43278093372407511, -275.9541996346974315, -334.1630939716773696 ) ) ;
#54796=CARTESIAN_POINT ( 'NONE',  ( -37.52009564963651655, -284.9148594880118708, -344.6087466678422970 ) ) ;
#54797=CARTESIAN_POINT ( 'NONE',  ( -64.60750629945529511, -275.8944384777469168, -338.8790562822850916 ) ) ;
#54798=DIRECTION ( 'NONE',  ( -1.000000000000000000, -0.000000000000000000, -0.000000000000000000 ) ) ;
#54799=CARTESIAN_POINT ( 'NONE',  ( 23.30033620924232807, -276.0611079736791567, -229.1467452166400562 ) ) ;
#54802=CIRCLE ( 'NONE', #66915, 0.5000000000000004441 ) ;
#54803=CARTESIAN_POINT ( 'NONE',  ( -92.96394086728045636, -280.0819476193443620, -217.2725849413230321 ) ) ;
#54804=EDGE_LOOP ( 'NONE', ( #25543, #52432, #71585, #74255 ) ) ;
#54806=CARTESIAN_POINT ( 'NONE',  ( -65.44162544547695859, -287.5491189129509166, -199.9859797679958433 ) ) ;
#54807=CARTESIAN_POINT ( 'NONE',  ( -78.04805593058895852, -294.8116770066197319, -331.2137146232465170 ) ) ;
#54808=CARTESIAN_POINT ( 'NONE',  ( -74.38550402990404109, -288.8800144851840059, -337.7636094896698182 ) ) ;
#54809=CARTESIAN_POINT ( 'NONE',  ( 21.15514057784789514, -285.1621201716123437, -225.0169491875583390 ) ) ;
#54810=CARTESIAN_POINT ( 'NONE',  ( 22.48110275398108016, -285.5316811332732527, -227.4195240120962467 ) ) ;
#54811=CARTESIAN_POINT ( 'NONE',  ( -109.6575680285130971, -288.5862398488591793, -286.1804893596330430 ) ) ;
#54812=CARTESIAN_POINT ( 'NONE',  ( -103.8517444957814888, -286.1755457617657044, -239.1995692458752387 ) ) ;
#54813=CARTESIAN_POINT ( 'NONE',  ( 21.92161414251100737, -274.1823983569975098, -316.3477975349532016 ) ) ;
#54814=CARTESIAN_POINT ( 'NONE',  ( 19.70156358983043532, -285.2598003058698737, -219.7608652349659337 ) ) ;
#54815=CARTESIAN_POINT ( 'NONE',  ( -35.90254134505045158, -300.0703241510347539, -195.3606186102793174 ) ) ;
#54816=CARTESIAN_POINT ( 'NONE',  ( 35.01258594108399791, -285.8140253493967293, -290.7770059657278807 ) ) ;
#54817=CARTESIAN_POINT ( 'NONE',  ( -37.01928345502811624, -280.9975414598524708, -197.1265325981078718 ) ) ;
#54818=CARTESIAN_POINT ( 'NONE',  ( 2.236991035479711787, -290.5239512990511912, -334.3248930398124799 ) ) ;
#54821=CARTESIAN_POINT ( 'NONE',  ( -76.31807526952506748, -297.4886794633707723, -335.1533949307752778 ) ) ;
#54822=CARTESIAN_POINT ( 'NONE',  ( -41.12734230361837007, -278.0043305825820994, -195.4567151489958974 ) ) ;
#54823=CARTESIAN_POINT ( 'NONE',  ( 6.412687804880273568, -291.8273387019003167, -207.1969481020532555 ) ) ;
#54824=CARTESIAN_POINT ( 'NONE',  ( -95.91167455816636789, -295.5770976640273489, -225.4406616544906967 ) ) ;
#54825=CARTESIAN_POINT ( 'NONE',  ( 35.91915802245630118, -280.3214849789204663, -276.8109756124551950 ) ) ;
#54826=CARTESIAN_POINT ( 'NONE',  ( 30.40655649460581245, -273.2227079598729347, -239.3901362487319204 ) ) ;
#54827=CARTESIAN_POINT ( 'NONE',  ( 34.81170932346955738, -295.0503653960419115, -284.3299756189863956 ) ) ;
#54828=CARTESIAN_POINT ( 'NONE',  ( -54.42813229853332757, -297.7662352645559167, -345.3683826091709648 ) ) ;
#54829=CARTESIAN_POINT ( 'NONE',  ( -110.9480689593987677, -295.2885518450696054, -250.0461612900226100 ) ) ;
#54830=CARTESIAN_POINT ( 'NONE',  ( 0.02243465603823597068, -292.8018751581251422, -336.5417622517857126 ) ) ;
#54831=CARTESIAN_POINT ( 'NONE',  ( -108.2890523582798608, -291.7190814596109476, -290.0896631170522255 ) ) ;
#54833=CARTESIAN_POINT ( 'NONE',  ( -37.56067507498378433, -292.8522121039181343, -197.1874975497974276 ) ) ;
#54835=CARTESIAN_POINT ( 'NONE',  ( -68.52923924434824698, -281.4800017822921063, -338.9736539246545135 ) ) ;
#54836=CARTESIAN_POINT ( 'NONE',  ( 22.58793393945703798, -292.9709258747196259, -228.6564952919479481 ) ) ;
#54837=CARTESIAN_POINT ( 'NONE',  ( -35.33602872409019113, -280.0766431042238764, -193.3741071519398815 ) ) ;
#54838=CARTESIAN_POINT ( 'NONE',  ( -63.90870195292774980, -283.0560537942198494, -342.6102612683880011 ) ) ;
#54839=CARTESIAN_POINT ( 'NONE',  ( -59.24958166259710879, -287.3360734146154414, -341.9699411778946683 ) ) ;
#54841=CARTESIAN_POINT ( 'NONE',  ( -69.65103336461976369, -278.1144435353747326, -201.2178877335352354 ) ) ;
#54842=CARTESIAN_POINT ( 'NONE',  ( 25.59014520486699240, -287.0550844105828219, -314.2823501210327208 ) ) ;
#54844=CARTESIAN_POINT ( 'NONE',  ( 35.50030252792328156, -294.9965954621784476, -258.4296724919660164 ) ) ;
#54845=CARTESIAN_POINT ( 'NONE',  ( -56.75665513531810547, -278.7228511356416334, -344.3188293972524434 ) ) ;
#54846=CARTESIAN_POINT ( 'NONE',  ( -81.29722343276812069, -279.1027718753659883, -211.9881145877385507 ) ) ;
#54847=CARTESIAN_POINT ( 'NONE',  ( 39.23730353364649659, -293.8255316677272617, -278.8927593026595559 ) ) ;
#54848=CARTESIAN_POINT ( 'NONE',  ( -89.46287041735449463, -281.8589296416707271, -325.1384387384256911 ) ) ;
#54850=CARTESIAN_POINT ( 'NONE',  ( 21.18905228942488961, -291.9947771703691615, -226.3434002977374462 ) ) ;
#54852=CARTESIAN_POINT ( 'NONE',  ( -103.4776497130817887, -295.0225600436410787, -234.8810185756578335 ) ) ;
#54856=CARTESIAN_POINT ( 'NONE',  ( 16.19997211966036588, -293.7737300012386186, -320.0730659892619201 ) ) ;
#54858=CARTESIAN_POINT ( 'NONE',  ( -53.28691492658257545, -289.3380690714490129, -200.3538533559491555 ) ) ;
#54859=CARTESIAN_POINT ( 'NONE',  ( -113.3829859678191383, -271.8922269560968061, -258.9585404145392431 ) ) ;
#54860=CARTESIAN_POINT ( 'NONE',  ( 14.33642407780962458, -278.9084983517965384, -214.8847126262412530 ) ) ;
#54862=CARTESIAN_POINT ( 'NONE',  ( 9.495554926013772601, -287.9963515147975954, -209.8667396451806155 ) ) ;
#54863=CARTESIAN_POINT ( 'NONE',  ( 20.35615608039524460, -288.0155285575916082, -315.1022395295304932 ) ) ;
#54865=CARTESIAN_POINT ( 'NONE',  ( -39.15560843221825849, -278.5954508057097314, -344.0321264650893340 ) ) ;
#54866=CARTESIAN_POINT ( 'NONE',  ( -107.3396433796828973, -294.9120854657339237, -244.2866028964509724 ) ) ;
#54867=CARTESIAN_POINT ( 'NONE',  ( -86.79376813557587411, -299.1131192690993998, -215.2932781742513555 ) ) ;
#54868=CARTESIAN_POINT ( 'NONE',  ( -97.21846944380278899, -276.7573155943226766, -312.8317798170293713 ) ) ;
#54870=CARTESIAN_POINT ( 'NONE',  ( -35.46828848052000183, -297.7417277859903493, -193.3823643072163634 ) ) ;
#54871=CARTESIAN_POINT ( 'NONE',  ( -61.70364572987922003, -291.2913674300612570, -340.7017876074841638 ) ) ;
#54872=CARTESIAN_POINT ( 'NONE',  ( 38.42833708171294660, -295.0440275860132715, -261.7953929749143640 ) ) ;
#54873=CARTESIAN_POINT ( 'NONE',  ( 202.9738562182569694, 291.9636489450776367, -53.99999999998589573 ) ) ;
#54875=CARTESIAN_POINT ( 'NONE',  ( -105.8090278388222174, -291.5465239389963585, -244.6026428687626151 ) ) ;
#54878=CARTESIAN_POINT ( 'NONE',  ( -101.4692718031482741, -297.7627846410916277, -227.8993312254676766 ) ) ;
#54879=CARTESIAN_POINT ( 'NONE',  ( -98.19807390327306962, -289.3017715993170782, -225.2083922436063972 ) ) ;
#54880=CARTESIAN_POINT ( 'NONE',  ( -37.61184835695555506, -298.3821352816740955, -193.3827358768863007 ) ) ;
#54883=CARTESIAN_POINT ( 'NONE',  ( 19.12434464653457766, -289.7762823793407847, -321.7059557083352956 ) ) ;
#54884=CARTESIAN_POINT ( 'NONE',  ( -111.2586520408596868, -286.6233781216988064, -305.9938812882205070 ) ) ;
#54885=CARTESIAN_POINT ( 'NONE',  ( -55.21838311417347001, -287.8219893343974718, -197.6407794336381585 ) ) ;
#54886=CARTESIAN_POINT ( 'NONE',  ( -67.83553264365225743, -288.0193613775954873, -340.4234650214762610 ) ) ;
#54887=CARTESIAN_POINT ( 'NONE',  ( -63.93500251437468762, -271.7044068885694514, -200.3985586211792054 ) ) ;
#54888=CARTESIAN_POINT ( 'NONE',  ( -21.65393943413130984, -276.1749814039736179, -197.5929356546862152 ) ) ;
#54889=CARTESIAN_POINT ( 'NONE',  ( -96.10205377780953029, -288.0003926761864932, -316.0822143136607565 ) ) ;
#54890=CARTESIAN_POINT ( 'NONE',  ( -101.0453745609532774, -279.8645374037464535, -311.4707963328471010 ) ) ;
#54894=CARTESIAN_POINT ( 'NONE',  ( -24.87639109164146589, -280.2156146946252306, -198.4332647501296094 ) ) ;
#54895=CARTESIAN_POINT ( 'NONE',  ( 7.211006969742085992, -280.0259070666188563, -212.3406256531423537 ) ) ;
#54896=CARTESIAN_POINT ( 'NONE',  ( 0.9048563303069437902, -277.6343780841357329, -336.8946121901996094 ) ) ;
#54897=CARTESIAN_POINT ( 'NONE',  ( 38.27340845060322749, -280.5022611584698211, -282.7052584524505505 ) ) ;
#54898=CARTESIAN_POINT ( 'NONE',  ( 200.9738562182569694, 293.6303156117443791, -53.99999999999359090 ) ) ;
#54899=CARTESIAN_POINT ( 'NONE',  ( 38.90534220976931579, -276.6106470413136549, -279.7073161796139402 ) ) ;
#54900=CARTESIAN_POINT ( 'NONE',  ( -96.41178290437866849, -274.7268709476192043, -222.0351007514593675 ) ) ;
#54901=CARTESIAN_POINT ( 'NONE',  ( 10.59707575819634329, -295.1948066931273615, -210.1954327657594490 ) ) ;
#54904=CARTESIAN_POINT ( 'NONE',  ( 16.19083254556992912, -287.9141173076805558, -220.2577290444759512 ) ) ;
#54905=CARTESIAN_POINT ( 'NONE',  ( 13.93663136718700457, -290.1050081977143691, -326.5083411736892458 ) ) ;
#54906=CARTESIAN_POINT ( 'NONE',  ( -107.8263138186721051, -289.6427314543595344, -289.9336064591886952 ) ) ;
#54907=CARTESIAN_POINT ( 'NONE',  ( -60.48543178116287322, -285.2676230270463407, -196.9305610713836927 ) ) ;
#54909=CARTESIAN_POINT ( 'NONE',  ( -8.196856329979501865, -281.0638363648741915, -338.1624343157080261 ) ) ;
#54910=CARTESIAN_POINT ( 'NONE',  ( 26.77464060336084017, -289.9187617785838142, -307.8788395695208919 ) ) ;
#54911=CARTESIAN_POINT ( 'NONE',  ( -83.24154654482278204, -282.1735572530329819, -328.0799892161239200 ) ) ;
#54912=CARTESIAN_POINT ( 'NONE',  ( -109.2437993338436826, -279.6680353039263309, -285.5707073681669499 ) ) ;
#54913=CARTESIAN_POINT ( 'NONE',  ( 7.623196754547683973, -276.9120515657534725, -328.0115805298017904 ) ) ;
#54914=CARTESIAN_POINT ( 'NONE',  ( -113.2704483345547288, -289.4794351917847166, -259.8326481741513589 ) ) ;
#54915=CARTESIAN_POINT ( 'NONE',  ( -67.13590330410211493, -286.4741778705596289, -199.5341155198975116 ) ) ;
#54916=CARTESIAN_POINT ( 'NONE',  ( -95.77393617394825753, -285.7210728215443964, -220.2292246856990516 ) ) ;
#54917=CARTESIAN_POINT ( 'NONE',  ( 33.65064803186798770, -281.9438259724282716, -287.4168490108671108 ) ) ;
#54920=CARTESIAN_POINT ( 'NONE',  ( -113.0164057037154777, -292.3656190973205753, -274.0549525888752669 ) ) ;
#54922=CARTESIAN_POINT ( 'NONE',  ( -61.51677111319927604, -290.4294952290104561, -197.7183827159624343 ) ) ;
#54923=CARTESIAN_POINT ( 'NONE',  ( 29.30513440849346196, -274.2014525121342672, -239.8804020983503165 ) ) ;
#54924=CARTESIAN_POINT ( 'NONE',  ( -114.2359538504407652, -295.9103309086441413, -269.5952650262510133 ) ) ;
#54925=CARTESIAN_POINT ( 'NONE',  ( -5.726795965617193396, -290.9554803908608278, -203.7799019042589350 ) ) ;
#54926=CARTESIAN_POINT ( 'NONE',  ( -94.74246341223364709, -294.1395260104930571, -317.1049815984326870 ) ) ;
#54927=AXIS2_PLACEMENT_3D ( 'NONE', #2557, #23855, #24313 ) ;
#54928=CARTESIAN_POINT ( 'NONE',  ( -56.15263018620973412, -290.5048547564448995, -341.3595668081164263 ) ) ;
#54931=CARTESIAN_POINT ( 'NONE',  ( -112.1934414860052840, -292.6128376651122949, -265.6475777042275013 ) ) ;
#54932=CARTESIAN_POINT ( 'NONE',  ( -9.174023103086078379, -290.4194269143868610, -200.6717328614652160 ) ) ;
#54933=CARTESIAN_POINT ( 'NONE',  ( -75.05734836781165598, -297.5546916495771939, -335.2027861620937301 ) ) ;
#54934=CARTESIAN_POINT ( 'NONE',  ( -91.70390561886109992, -286.1946121870005868, -221.2135908675137728 ) ) ;
#54935=CARTESIAN_POINT ( 'NONE',  ( 3.258994510386305166, -296.5085695020325147, -333.6807072992319831 ) ) ;
#54937=CARTESIAN_POINT ( 'NONE',  ( -13.60501259672264496, -276.3386887066903341, -198.8420543268857159 ) ) ;
#54938=CARTESIAN_POINT ( 'NONE',  ( -8.050736783225303839, -275.4718456513494971, -341.1570214346750163 ) ) ;
#54939=CARTESIAN_POINT ( 'NONE',  ( -43.26708147556938400, -297.1764333316074840, -193.6983029191631829 ) ) ;
#54940=CARTESIAN_POINT ( 'NONE',  ( 36.65648359150822699, -273.7725179426865907, -268.8635141839382641 ) ) ;
#54941=CARTESIAN_POINT ( 'NONE',  ( -43.85315350263300616, -278.0491970760363074, -196.1552225057391752 ) ) ;
#54942=CARTESIAN_POINT ( 'NONE',  ( -76.79050176104948378, -274.7160357706691229, -208.4666711062203888 ) ) ;
#54943=CARTESIAN_POINT ( 'NONE',  ( 2.129285921777238411, -273.1445538854864026, -204.9344601681925155 ) ) ;
#54946=CARTESIAN_POINT ( 'NONE',  ( -71.74996550566946496, -298.3880240043511094, -205.7816262832244263 ) ) ;
#54949=CARTESIAN_POINT ( 'NONE',  ( -40.29998282908324825, -287.1092485472597104, -345.6710339318566412 ) ) ;
#54950=CARTESIAN_POINT ( 'NONE',  ( 9.486706258851251405, -274.5501558829931810, -214.2940245204525240 ) ) ;
#54952=CARTESIAN_POINT ( 'NONE',  ( 3.180135298615699657, -288.5241132358754044, -335.8987058422258656 ) ) ;
#54953=CARTESIAN_POINT ( 'NONE',  ( -36.09144325118830210, -288.7036326836868625, -347.3429271837919146 ) ) ;
#54954=CARTESIAN_POINT ( 'NONE',  ( -86.41075002089942814, -299.3551486533382331, -213.1028438763793815 ) ) ;
#54955=CARTESIAN_POINT ( 'NONE',  ( -50.82594392346678092, -293.2246655479536912, -343.9695658193610370 ) ) ;
#54956=CARTESIAN_POINT ( 'NONE',  ( 30.92898429233507684, -281.2047961234276272, -305.6211870235620154 ) ) ;
#54958=CARTESIAN_POINT ( 'NONE',  ( 22.31120660474435624, -278.9296226006674146, -224.8811695122272738 ) ) ;
#54961=CARTESIAN_POINT ( 'NONE',  ( -15.74940643767814841, -287.5615481272288889, -340.5633772645647355 ) ) ;
#54964=CARTESIAN_POINT ( 'NONE',  ( -69.86239269815402508, -289.6238236197082188, -202.7643578217271170 ) ) ;
#54965=CARTESIAN_POINT ( 'NONE',  ( -69.81374712839919994, -275.1366480142143587, -204.2077059900510392 ) ) ;
#54966=CARTESIAN_POINT ( 'NONE',  ( 36.41147801202088630, -282.7247469650839093, -250.3346821671716498 ) ) ;
#54967=CARTESIAN_POINT ( 'NONE',  ( -62.27649911082106371, -295.7495263444196780, -199.2509035166758338 ) ) ;
#54968=CARTESIAN_POINT ( 'NONE',  ( -110.0957674051256845, -284.4731720123492664, -276.3482453945421753 ) ) ;
#54969=CARTESIAN_POINT ( 'NONE',  ( -67.31398096410767096, -275.0765042358539745, -203.1384047884904760 ) ) ;
#54970=CARTESIAN_POINT ( 'NONE',  ( 32.21214304518407090, -276.0526193022728876, -247.5075887888366992 ) ) ;
#54971=CARTESIAN_POINT ( 'NONE',  ( -65.79332031218706334, -285.4244470023178337, -339.7687797464978416 ) ) ;
#54972=EDGE_CURVE ( 'NONE', #66639, #21957, #30334, .T. ) ;
#54973=CARTESIAN_POINT ( 'NONE',  ( -106.5939053662181664, -271.7909678117702583, -246.3120401825525221 ) ) ;
#54975=CARTESIAN_POINT ( 'NONE',  ( 204.7092198302316035, 294.9664581756286452, -54.00000000004281731 ) ) ;
#54976=CARTESIAN_POINT ( 'NONE',  ( 37.42245399029074804, -293.1550338909091806, -251.9404430900545435 ) ) ;
#54977=CARTESIAN_POINT ( 'NONE',  ( -75.58395531270943479, -287.5190959269237965, -206.2566975345147284 ) ) ;
#54979=CARTESIAN_POINT ( 'NONE',  ( 40.64545035920995986, -279.2666405000204009, -288.1938231032136741 ) ) ;
#54980=CARTESIAN_POINT ( 'NONE',  ( -114.0490556539642597, -277.8055653820600241, -265.8733091314261401 ) ) ;
#54981=CARTESIAN_POINT ( 'NONE',  ( -112.3494774162785035, -288.7814145140571327, -283.8615341361522155 ) ) ;
#54982=CARTESIAN_POINT ( 'NONE',  ( -98.09304339416746643, -285.4960014812526197, -312.1631152127524160 ) ) ;
#54983=CARTESIAN_POINT ( 'NONE',  ( -67.19106464212329399, -279.2091295583560964, -338.0884348761078968 ) ) ;
#54984=CARTESIAN_POINT ( 'NONE',  ( -112.4227553300736275, -286.1597201042796996, -255.8924558512456429 ) ) ;
#54985=CARTESIAN_POINT ( 'NONE',  ( -74.00839501187840597, -282.3454516190755044, -334.0011452165243213 ) ) ;
#54986=CARTESIAN_POINT ( 'NONE',  ( -68.15052461716483378, -281.6477724934836147, -201.9671904972286995 ) ) ;
#54987=CARTESIAN_POINT ( 'NONE',  ( -46.88310250723962724, -274.1008436232017402, -193.9545629945613427 ) ) ;
#54988=CARTESIAN_POINT ( 'NONE',  ( -37.12909664450568670, -276.8828453939410679, -347.3738831291669271 ) ) ;
#54990=CARTESIAN_POINT ( 'NONE',  ( -87.44143037816654385, -297.6778042941705280, -325.4186444838368857 ) ) ;
#54995=CARTESIAN_POINT ( 'NONE',  ( -112.1658791884912461, -294.8440539516494709, -258.3775054057362013 ) ) ;
#54996=CARTESIAN_POINT ( 'NONE',  ( 7.613327878650325786, -275.9275156067258763, -328.0192763208009410 ) ) ;
#54998=CARTESIAN_POINT ( 'NONE',  ( -96.63852159007261378, -274.4118757709899796, -221.8442972438961931 ) ) ;
#54999=CARTESIAN_POINT ( 'NONE',  ( 36.46424283905096786, -289.3927457632027540, -276.5439795133319762 ) ) ;
#55000=CARTESIAN_POINT ( 'NONE',  ( -93.16889471955472857, -297.3564947689035307, -322.3998925472031374 ) ) ;
#55001=CARTESIAN_POINT ( 'NONE',  ( -3.390892033970570374, -295.8190153851442119, -339.0440637491524285 ) ) ;
#55002=CARTESIAN_POINT ( 'NONE',  ( -82.86398811087624949, -293.4285347695969790, -210.9006660024705297 ) ) ;
#55003=CARTESIAN_POINT ( 'NONE',  ( -7.239164970448359604, -278.4477156171212755, -201.8353064887004393 ) ) ;
#55005=CARTESIAN_POINT ( 'NONE',  ( -66.65891021632147329, -281.5852767898416573, -201.9234150036206472 ) ) ;
#55006=CARTESIAN_POINT ( 'NONE',  ( -111.2369820726292602, -294.5103544024182725, -279.7639477784231872 ) ) ;
#55007=CARTESIAN_POINT ( 'NONE',  ( -104.6753602359658970, -285.9562541416623276, -305.2099924881246125 ) ) ;
#55008=CARTESIAN_POINT ( 'NONE',  ( 35.06235889184210919, -286.6243781957236934, -281.9248511678536033 ) ) ;
#55009=CARTESIAN_POINT ( 'NONE',  ( -105.9390882850879336, -263.2164998017994435, -317.4572233070413745 ) ) ;
#55011=CARTESIAN_POINT ( 'NONE',  ( -67.55257157191294937, -285.3112430140916445, -203.8826197033241385 ) ) ;
#55013=CARTESIAN_POINT ( 'NONE',  ( -5.570976448279924220, -283.7236297573737147, -340.1616453998773864 ) ) ;
#55015=CARTESIAN_POINT ( 'NONE',  ( -92.93263885425096760, -273.5588659936238400, -222.9948510194683706 ) ) ;
#55016=CARTESIAN_POINT ( 'NONE',  ( 1.334521340504313036, -285.3516813282454336, -204.2235567117757853 ) ) ;
#55018=CARTESIAN_POINT ( 'NONE',  ( -36.76639190577337502, -281.0004650638578028, -193.5855615632846991 ) ) ;
#55020=CARTESIAN_POINT ( 'NONE',  ( -111.7302002237050544, -280.2868291554520397, -253.3593883797751118 ) ) ;
#55021=CARTESIAN_POINT ( 'NONE',  ( 25.09262785313039146, -282.4829049339294897, -315.4134738469486479 ) ) ;
#55022=CARTESIAN_POINT ( 'NONE',  ( -102.0172624299487154, -282.4809262143061233, -239.1787733560258289 ) ) ;
#55023=CARTESIAN_POINT ( 'NONE',  ( -113.0733666116212106, -274.4133621447950873, -270.3848156438984915 ) ) ;
#55025=CARTESIAN_POINT ( 'NONE',  ( 25.31494228580528727, -276.9991902721702104, -229.4444516038402924 ) ) ;
#55026=CARTESIAN_POINT ( 'NONE',  ( 83.91869577041705952, 83.53290714828214902, -302.0006688339001926 ) ) ;
#55028=CARTESIAN_POINT ( 'NONE',  ( 10.34629288835905925, -278.7336583536934995, -212.8680968326108882 ) ) ;
#55029=CARTESIAN_POINT ( 'NONE',  ( 29.99047499235947001, -294.8505367082642579, -235.0292724524110781 ) ) ;
#55030=CARTESIAN_POINT ( 'NONE',  ( -41.05267997585957573, -294.4486358492787303, -343.3813824908961578 ) ) ;
#55031=CARTESIAN_POINT ( 'NONE',  ( -88.60381308502861941, -290.8630468635778357, -212.9875815893325637 ) ) ;
#55032=FACE_OUTER_BOUND ( 'NONE', #53654, .T. ) ;
#55033=CARTESIAN_POINT ( 'NONE',  ( -97.81931182513881140, -294.4987277959338599, -317.0629892348457020 ) ) ;
#55034=CARTESIAN_POINT ( 'NONE',  ( 25.64399040087455006, -285.4278823042268414, -231.9001871203971064 ) ) ;
#55035=CARTESIAN_POINT ( 'NONE',  ( 30.63039618845291656, -295.8073729279712438, -300.2050386357032039 ) ) ;
#55036=CARTESIAN_POINT ( 'NONE',  ( 31.85814902199712861, -286.5643272006735742, -295.1123675489823199 ) ) ;
#55037=CARTESIAN_POINT ( 'NONE',  ( -83.97361805691599557, -286.7113696298605419, -213.4908662941040234 ) ) ;
#55038=CARTESIAN_POINT ( 'NONE',  ( 30.68483988825011366, -294.0317792577080809, -234.6769264103842829 ) ) ;
#55039=CARTESIAN_POINT ( 'NONE',  ( -32.13506353297257334, -283.4770510601232445, -343.2368984386381499 ) ) ;
#55040=CARTESIAN_POINT ( 'NONE',  ( -111.5876131819561721, -295.1093106901842589, -289.2702317953996953 ) ) ;
#55042=CARTESIAN_POINT ( 'NONE',  ( -109.3261651164391424, -291.6973232722439775, -243.3320156031787747 ) ) ;
#55043=CARTESIAN_POINT ( 'NONE',  ( -111.9364526678255203, -291.2810858828339065, -251.4626154007349896 ) ) ;
#55044=CARTESIAN_POINT ( 'NONE',  ( 21.96293194122219461, -288.3138876279226110, -312.9282487249849396 ) ) ;
#55047=CARTESIAN_POINT ( 'NONE',  ( -112.9988147667955189, -298.3500086414654220, -275.2831235803675440 ) ) ;
#55048=CARTESIAN_POINT ( 'NONE',  ( -112.4015799369000206, -295.4242340436867948, -255.4846087154301699 ) ) ;
#55049=CARTESIAN_POINT ( 'NONE',  ( -32.93692382291894916, -279.1677519355563390, -197.2584067186867287 ) ) ;
#55051=CARTESIAN_POINT ( 'NONE',  ( 26.09738068237256314, -274.4845862887783596, -226.8060521823317401 ) ) ;
#55052=CARTESIAN_POINT ( 'NONE',  ( -100.4809364185774143, -295.5511897397036023, -232.2600215203199809 ) ) ;
#55053=CARTESIAN_POINT ( 'NONE',  ( -26.82347436592075596, -278.7773891892311440, -343.8473915668690779 ) ) ;
#55054=CARTESIAN_POINT ( 'NONE',  ( 35.92235194768895923, -273.8510113750921278, -282.6395878273263520 ) ) ;
#55055=CARTESIAN_POINT ( 'NONE',  ( -103.1172240140658403, -297.3167534111528880, -303.0444805387761562 ) ) ;
#55056=CARTESIAN_POINT ( 'NONE',  ( -79.91869786696278766, -298.5404709321466044, -210.6834392714524711 ) ) ;
#55058=CARTESIAN_POINT ( 'NONE',  ( -104.5576414103637575, -298.6222694634119534, -234.3540368884742122 ) ) ;
#55059=CARTESIAN_POINT ( 'NONE',  ( -37.57576512040230909, -296.0490714457672539, -195.1948114014585940 ) ) ;
#55060=CARTESIAN_POINT ( 'NONE',  ( -66.61249707010439636, -292.3097151932946076, -203.3752006952508680 ) ) ;
#55061=CARTESIAN_POINT ( 'NONE',  ( -109.5202016453131932, -288.9383771518809567, -284.7657633322738775 ) ) ;
#55063=CARTESIAN_POINT ( 'NONE',  ( 34.12942102622687912, -276.4077785896535602, -298.9899697542564923 ) ) ;
#55064=CARTESIAN_POINT ( 'NONE',  ( -99.28160066503373571, -273.2520370819111690, -231.7288940500819194 ) ) ;
#55065=CARTESIAN_POINT ( 'NONE',  ( 20.68760796642643385, -282.8716505531958205, -222.2881920403038407 ) ) ;
#55066=CARTESIAN_POINT ( 'NONE',  ( -5.675020661157632595, -281.3291717171906043, -340.0067903960325566 ) ) ;
#55067=CARTESIAN_POINT ( 'NONE',  ( -22.96610244330243589, -276.2216018292771764, -345.9576354803714366 ) ) ;
#55068=CARTESIAN_POINT ( 'NONE',  ( -106.3294106731240731, -283.4240847983955405, -294.8697389306987020 ) ) ;
#55069=CARTESIAN_POINT ( 'NONE',  ( 37.78658544189189428, -279.5827599667654226, -272.7630195029399829 ) ) ;
#55071=CARTESIAN_POINT ( 'NONE',  ( -89.64833776897799567, -271.8711971205275404, -218.5982879261818539 ) ) ;
#55072=CARTESIAN_POINT ( 'NONE',  ( -67.33731659946909076, -279.4456402257029026, -339.1153919793142677 ) ) ;
#55075=CARTESIAN_POINT ( 'NONE',  ( -59.82656767513203988, -296.0047597183929042, -197.7225550755167944 ) ) ;
#55077=CARTESIAN_POINT ( 'NONE',  ( -110.9920390383823161, -280.3590449780327845, -285.4464746146342691 ) ) ;
#55078=CARTESIAN_POINT ( 'NONE',  ( 18.79913333761682281, -272.8596833547986193, -220.5527788359568717 ) ) ;
#55080=CARTESIAN_POINT ( 'NONE',  ( -100.2072239040783614, -285.9089413896007841, -312.3744031281288471 ) ) ;
#55084=CARTESIAN_POINT ( 'NONE',  ( 37.52703297763829227, -285.6191223741221847, -275.5897078622135723 ) ) ;
#55086=CARTESIAN_POINT ( 'NONE',  ( 6.286712081043673628, -293.2400247341555541, -329.4472578727649079 ) ) ;
#55087=CARTESIAN_POINT ( 'NONE',  ( 8.728284001572998108, -286.5524324248123662, -328.5712720771620070 ) ) ;
#55088=CARTESIAN_POINT ( 'NONE',  ( -96.12512592106646991, -239.9971452530988358, -342.0757611934672582 ) ) ;
#55089=CARTESIAN_POINT ( 'NONE',  ( -91.47217133725644089, -295.2819183495281550, -218.3744672509484133 ) ) ;
#55090=CARTESIAN_POINT ( 'NONE',  ( -3.776712206258508342, -284.9668114387247329, -201.8186270729092087 ) ) ;
#55091=CARTESIAN_POINT ( 'NONE',  ( 32.72982709204060825, -282.8462518437090694, -247.0394153964454347 ) ) ;
#55092=CARTESIAN_POINT ( 'NONE',  ( 28.86780280704394386, -280.2834824471888737, -307.7547008041527192 ) ) ;
#55093=CARTESIAN_POINT ( 'NONE',  ( -8.218492891473735185, -288.6599682130220117, -337.3542252515497921 ) ) ;
#55094=CONICAL_SURFACE ( 'NONE', #59643, 1.898405138727909947, 0.09862129276975308001 ) ;
#55096=CARTESIAN_POINT ( 'NONE',  ( -51.96203921225311007, -281.2867868616741021, -198.1867062476765113 ) ) ;
#55097=CARTESIAN_POINT ( 'NONE',  ( 0.4746802127685552097, -281.3725421214461448, -207.6724285456314476 ) ) ;
#55098=CARTESIAN_POINT ( 'NONE',  ( 38.05711380274217248, -289.5466105002838617, -271.5007028480964095 ) ) ;
#55100=CIRCLE ( 'NONE', #79318, 5.654241149514405151 ) ;
#55101=CARTESIAN_POINT ( 'NONE',  ( -46.88099868354511557, -273.9341904422645939, -193.9543003347235413 ) ) ;
#55102=CARTESIAN_POINT ( 'NONE',  ( -85.73257901406893211, -291.7052918818141052, -327.2639039531634921 ) ) ;
#55104=CARTESIAN_POINT ( 'NONE',  ( -99.86837403722181250, -298.4090924074129703, -320.2651865833026363 ) ) ;
#55106=CARTESIAN_POINT ( 'NONE',  ( 36.37920228237386056, -273.7399587383893049, -285.0327565243341041 ) ) ;
#55108=CARTESIAN_POINT ( 'NONE',  ( 151.9709352735115147, -299.5541904835127980, -197.2582414438974183 ) ) ;
#55109=CARTESIAN_POINT ( 'NONE',  ( -110.0427152187716615, -294.6617036427807079, -293.2303160266133091 ) ) ;
#55110=CARTESIAN_POINT ( 'NONE',  ( -57.91611124994465598, -297.2867469880741851, -200.2563246479271868 ) ) ;
#55111=CARTESIAN_POINT ( 'NONE',  ( 23.33163633881805055, -289.6495488696513121, -312.2098436545985010 ) ) ;
#55113=CARTESIAN_POINT ( 'NONE',  ( -81.20895526196396474, -285.4172873167271405, -330.0372665317050291 ) ) ;
#55114=CARTESIAN_POINT ( 'NONE',  ( -90.39002824820366300, -292.7445804157604812, -215.2923836465211878 ) ) ;
#55115=CARTESIAN_POINT ( 'NONE',  ( -71.67008800354003029, -290.8114184341671375, -338.7340662914699578 ) ) ;
#55116=CARTESIAN_POINT ( 'NONE',  ( -84.93619388626592581, -287.3962458661115988, -212.3301429755593688 ) ) ;
#55117=CARTESIAN_POINT ( 'NONE',  ( -96.81878921080129885, -279.3759210904946144, -221.4378955750481452 ) ) ;
#55118=CARTESIAN_POINT ( 'NONE',  ( -109.4317407034382796, -294.9238296613741568, -247.5529225358245924 ) ) ;
#55119=CARTESIAN_POINT ( 'NONE',  ( 19.78208454764835622, -282.0872807508259825, -322.0712179649178211 ) ) ;
#55120=CARTESIAN_POINT ( 'NONE',  ( 22.46244029927251873, -276.8065720072918907, -226.3800962795182272 ) ) ;
#55121=CARTESIAN_POINT ( 'NONE',  ( -6.941161984400275209, -279.1233781216987495, -333.4151289067050357 ) ) ;
#55123=CARTESIAN_POINT ( 'NONE',  ( -103.9019338409810018, -276.2157459506518649, -306.5556032828854995 ) ) ;
#55125=CARTESIAN_POINT ( 'NONE',  ( 29.03120913537884817, -280.6467076401698932, -239.7009358238125571 ) ) ;
#55126=CARTESIAN_POINT ( 'NONE',  ( -113.8153468472678469, -279.8131504042410143, -265.9125142601948824 ) ) ;
#55127=CARTESIAN_POINT ( 'NONE',  ( -106.4620324521435037, -284.0406938643907893, -236.9665095601148721 ) ) ;
#55128=CARTESIAN_POINT ( 'NONE',  ( 19.23693497491149174, -294.6436100630608053, -222.6449565105515660 ) ) ;
#55129=CARTESIAN_POINT ( 'NONE',  ( 38.51879647238281024, -277.0547134257152493, -262.6409225931761853 ) ) ;
#55130=CARTESIAN_POINT ( 'NONE',  ( -0.2989814327212445000, -275.8492501569752449, -203.4049401091162395 ) ) ;
#55132=CARTESIAN_POINT ( 'NONE',  ( -24.33168797528820448, -276.7148708051191761, -342.2438959058888486 ) ) ;
#55133=CARTESIAN_POINT ( 'NONE',  ( -108.4568213082627892, -298.8558147294182277, -246.9014283893224047 ) ) ;
#55134=CARTESIAN_POINT ( 'NONE',  ( -72.00537838965749415, -283.5925013780081940, -204.0402476723845950 ) ) ;
#55135=CARTESIAN_POINT ( 'NONE',  ( 39.42030021258337058, -293.1466395762262209, -264.5870730265211250 ) ) ;
#55136=CARTESIAN_POINT ( 'NONE',  ( 37.23628636940647141, -288.9538419730869805, -254.6594656673554766 ) ) ;
#55138=CARTESIAN_POINT ( 'NONE',  ( 20.43497337705931471, -291.8389277840722684, -225.2178247258592023 ) ) ;
#55140=CARTESIAN_POINT ( 'NONE',  ( -36.36750755057224183, -290.6388760579702648, -193.9436219705045232 ) ) ;
#55141=CARTESIAN_POINT ( 'NONE',  ( -12.24895511555226513, -292.0543827685047518, -201.7328722968619275 ) ) ;
#55143=CARTESIAN_POINT ( 'NONE',  ( 36.39020323517412692, -288.3641411897697822, -249.0753066624780274 ) ) ;
#55144=CARTESIAN_POINT ( 'NONE',  ( -110.1800361393731862, -278.9535340963604426, -265.1973699433982006 ) ) ;
#55146=CARTESIAN_POINT ( 'NONE',  ( -41.94082350121679781, -294.0290266843757649, -346.9661620694162707 ) ) ;
#55147=CARTESIAN_POINT ( 'NONE',  ( -105.3458319326085046, -285.6689643164045265, -234.3479059576969519 ) ) ;
#55148=CARTESIAN_POINT ( 'NONE',  ( 38.53529940281632804, -287.7221113214654906, -257.3057220293805472 ) ) ;
#55149=CARTESIAN_POINT ( 'NONE',  ( -24.05748596012324114, -283.2110619448767466, -342.1637442620149159 ) ) ;
#55150=CARTESIAN_POINT ( 'NONE',  ( 199.7395823140011828, 289.5256457063815105, -97.52092915841859622 ) ) ;
#55151=CARTESIAN_POINT ( 'NONE',  ( 101.7873421534306999, 116.6550764272915472, -281.9818386274820909 ) ) ;
#55152=CARTESIAN_POINT ( 'NONE',  ( 63.99139254834007318, 46.87924742655182087, -315.4201083341205845 ) ) ;
#55153=CARTESIAN_POINT ( 'NONE',  ( 34.78657350390782454, -274.5870674316201416, -258.0345504581135856 ) ) ;
#55154=CARTESIAN_POINT ( 'NONE',  ( -3.737971832439035413, -275.5181263251067776, -335.5149015954532388 ) ) ;
#55155=CARTESIAN_POINT ( 'NONE',  ( -62.81875398917058106, -297.2368315542349819, -197.7632762122106556 ) ) ;
#55156=CARTESIAN_POINT ( 'NONE',  ( -110.3257684885215753, -272.2967757702207905, -283.7855995824492652 ) ) ;
#55157=CARTESIAN_POINT ( 'NONE',  ( 39.12969167563818473, -274.2832489175389696, -274.0370798290085759 ) ) ;
#55158=CARTESIAN_POINT ( 'NONE',  ( -93.69976746502780429, -274.9854953453994426, -222.3650707476377022 ) ) ;
#55160=CARTESIAN_POINT ( 'NONE',  ( 7.805039230333843392, -299.5456763218493847, -193.5893858898706412 ) ) ;
#55161=CARTESIAN_POINT ( 'NONE',  ( 31.02996916658182514, -287.6993974261896483, -244.4636616652207692 ) ) ;
#55162=CARTESIAN_POINT ( 'NONE',  ( -84.07886516745874417, -296.4786911568550067, -331.4183278053247932 ) ) ;
#55163=CARTESIAN_POINT ( 'NONE',  ( -102.2678288998948517, -297.5859989288934457, -229.0800726243258509 ) ) ;
#55164=CARTESIAN_POINT ( 'NONE',  ( 20.52450394613299167, -294.3453701634355753, -314.8844214141962539 ) ) ;
#55167=CARTESIAN_POINT ( 'NONE',  ( 35.50400189142177254, -277.7290717748321640, -290.4797439349166552 ) ) ;
#55169=CARTESIAN_POINT ( 'NONE',  ( 22.83111133083752975, -280.4171768318689146, -222.3947883097530109 ) ) ;
#55171=CARTESIAN_POINT ( 'NONE',  ( -64.40898970142997371, -278.3554151877087293, -338.4647322349119918 ) ) ;
#55172=CARTESIAN_POINT ( 'NONE',  ( 37.73811906032817376, -277.4648157605892607, -282.3964475737441262 ) ) ;
#55173=CARTESIAN_POINT ( 'NONE',  ( -109.8645536581271642, -276.3101747354804161, -290.8267604190215252 ) ) ;
#55174=CARTESIAN_POINT ( 'NONE',  ( -71.72026397244610507, -298.2366291088175672, -205.8332807532226241 ) ) ;
#55175=TOROIDAL_SURFACE ( 'NONE', #32531, 5.654241149514406040, 0.5000000000000000000 ) ;
#55176=CARTESIAN_POINT ( 'NONE',  ( -53.29465604947596091, -293.8353422073069510, -342.2527766614713300 ) ) ;
#55178=CARTESIAN_POINT ( 'NONE',  ( 36.11508859233749291, -281.7567971005397567, -247.4782183821648118 ) ) ;
#55179=CARTESIAN_POINT ( 'NONE',  ( -89.08432308948820832, -277.9712187743338632, -321.9275661965899644 ) ) ;
#55181=CARTESIAN_POINT ( 'NONE',  ( -8.435081188999458135, -287.3664129927677777, -341.2110567234966538 ) ) ;
#55182=CARTESIAN_POINT ( 'NONE',  ( -2.260155546028384421, -276.5166566964427943, -204.0717079610543294 ) ) ;
#55184=CARTESIAN_POINT ( 'NONE',  ( -39.97410885093962207, -288.2831062310106631, -343.5249103598009128 ) ) ;
#55185=CARTESIAN_POINT ( 'NONE',  ( -102.4277797940218591, -284.4377262680526428, -229.4085231909915592 ) ) ;
#55186=CARTESIAN_POINT ( 'NONE',  ( 16.00510946426042125, -279.0607456820833931, -218.9839609021265687 ) ) ;
#55187=CARTESIAN_POINT ( 'NONE',  ( 3.042385127813834966, -279.1804755766375479, -208.7816694181454693 ) ) ;
#55188=CARTESIAN_POINT ( 'NONE',  ( -109.4949100655157395, -282.3950161994323480, -288.6703641864324368 ) ) ;
#55189=CARTESIAN_POINT ( 'NONE',  ( 0.8113929982533748531, -288.5607796618269845, -205.7313282214225296 ) ) ;
#55190=CARTESIAN_POINT ( 'NONE',  ( -110.7488192859057392, -279.7893912150559572, -267.9102303766407545 ) ) ;
#55192=CARTESIAN_POINT ( 'NONE',  ( -78.51822587480140214, -293.4984325618755179, -207.6133449737126853 ) ) ;
#55193=CARTESIAN_POINT ( 'NONE',  ( -86.45751392806090507, -275.9628475672048467, -328.4093815558453002 ) ) ;
#55194=CARTESIAN_POINT ( 'NONE',  ( -32.40540072151409845, -277.6398290439803418, -343.3462319723126370 ) ) ;
#55195=CARTESIAN_POINT ( 'NONE',  ( -105.3361541654581117, -286.1318357357983473, -302.4045672914245984 ) ) ;
#55197=EDGE_CURVE ( 'NONE', #33611, #55253, #54515, .T. ) ;
#55199=CARTESIAN_POINT ( 'NONE',  ( -112.6746729194045855, -292.3895489858472843, -276.8546433482543421 ) ) ;
#55200=CARTESIAN_POINT ( 'NONE',  ( -96.92632140702052368, -295.1757803319283084, -224.7917452346152913 ) ) ;
#55201=CARTESIAN_POINT ( 'NONE',  ( 35.79092297157611569, -287.0464164546436905, -293.9360678017284840 ) ) ;
#55203=CARTESIAN_POINT ( 'NONE',  ( 34.60755553167483356, -274.0398199433121249, -255.3146863642739675 ) ) ;
#55204=CARTESIAN_POINT ( 'NONE',  ( 2.208194918090676584, -292.6563584883252815, -333.2445250748014018 ) ) ;
#55207=CARTESIAN_POINT ( 'NONE',  ( -36.36759647675409468, -290.5440417597841929, -194.0477511856339277 ) ) ;
#55208=CARTESIAN_POINT ( 'NONE',  ( -79.78585596363124921, -287.0681116616775626, -209.9250792897136648 ) ) ;
#55209=CARTESIAN_POINT ( 'NONE',  ( 37.67091937069337604, -285.9497574773290012, -282.8081316248267854 ) ) ;
#55210=CARTESIAN_POINT ( 'NONE',  ( -79.66286394741386800, -286.8932837217631686, -210.0964393025636241 ) ) ;
#55212=CARTESIAN_POINT ( 'NONE',  ( -70.06380692778058972, -286.4125189212716123, -204.9111776814588950 ) ) ;
#55213=CARTESIAN_POINT ( 'NONE',  ( 33.88938516473130846, -295.2135217279840163, -245.6159439202195074 ) ) ;
#55214=CARTESIAN_POINT ( 'NONE',  ( 25.74204973801777996, -273.0746986587453762, -228.7707981888274560 ) ) ;
#55215=CARTESIAN_POINT ( 'NONE',  ( 39.60248571057819333, -275.9314387767858534, -274.0387203528847522 ) ) ;
#55216=CARTESIAN_POINT ( 'NONE',  ( -34.98044797458204869, -290.1614090621051787, -194.8251137098301626 ) ) ;
#55217=CARTESIAN_POINT ( 'NONE',  ( -88.93144521210125220, -279.3505833085660583, -213.1990833602177986 ) ) ;
#55218=CARTESIAN_POINT ( 'NONE',  ( -58.85880352909613578, -297.3117773647936701, -341.8374151835903945 ) ) ;
#55221=CARTESIAN_POINT ( 'NONE',  ( -68.97210693730590947, -284.3120884346226944, -204.0090065468893954 ) ) ;
#55222=CARTESIAN_POINT ( 'NONE',  ( -79.35017544545200963, -275.7650988312102527, -331.6295543714248879 ) ) ;
#55223=CARTESIAN_POINT ( 'NONE',  ( 21.32717738862364953, -278.9096077384258479, -223.6184964271196804 ) ) ;
#55225=CARTESIAN_POINT ( 'NONE',  ( 4.499316900309763056, -273.0851240053311244, -206.4859018074274672 ) ) ;
#55226=CARTESIAN_POINT ( 'NONE',  ( -101.9508798439227490, -277.4355544977078694, -304.5597519363249717 ) ) ;
#55227=CARTESIAN_POINT ( 'NONE',  ( -39.69193781160541334, -296.6022915896484164, -344.0295160471929421 ) ) ;
#55228=CARTESIAN_POINT ( 'NONE',  ( -6.342656464704358399, -279.3702204652519185, -200.2002566725798545 ) ) ;
#55229=CARTESIAN_POINT ( 'NONE',  ( -50.50176172447309852, -296.1656045496982301, -342.4043079885302632 ) ) ;
#55230=CARTESIAN_POINT ( 'NONE',  ( -40.43718541074416351, -299.3293050105615976, -193.8651226438979620 ) ) ;
#55231=CARTESIAN_POINT ( 'NONE',  ( -99.29617458852614220, -272.7521564427878502, -231.7123071202326514 ) ) ;
#55232=CARTESIAN_POINT ( 'NONE',  ( -71.14431879194852115, -293.6060966457828272, -203.4105121301606971 ) ) ;
#55233=CARTESIAN_POINT ( 'NONE',  ( -87.75154436182388906, -285.5374847025777854, -212.0853087964289898 ) ) ;
#55234=CARTESIAN_POINT ( 'NONE',  ( 34.56529314332229319, -273.3844938012794046, -246.3274069948136002 ) ) ;
#55235=CARTESIAN_POINT ( 'NONE',  ( -57.29294578360175905, -289.1358991989440597, -344.7865657775103614 ) ) ;
#55236=CARTESIAN_POINT ( 'NONE',  ( -35.65024809727083266, -282.0533365829164154, -195.7227977055770509 ) ) ;
#55237=CARTESIAN_POINT ( 'NONE',  ( 30.69935905039540458, -286.9738217597354151, -297.5869968447987048 ) ) ;
#55238=CARTESIAN_POINT ( 'NONE',  ( -34.99674505633289812, -290.0814155857904666, -195.3849731050563605 ) ) ;
#55239=VERTEX_POINT ( 'NONE', #26708 ) ;
#55240=CARTESIAN_POINT ( 'NONE',  ( 196.7899183121812712, 289.3460118731243824, -81.74456998406768093 ) ) ;
#55241=CARTESIAN_POINT ( 'NONE',  ( -18.46364438118356688, -288.3100947372988685, -340.9942502644269666 ) ) ;
#55242=CARTESIAN_POINT ( 'NONE',  ( -4.254362200211457612, -283.5678479515829054, -339.6435096994434844 ) ) ;
#55243=CARTESIAN_POINT ( 'NONE',  ( -72.05511189597812916, -290.6632161082450807, -201.8790591540609398 ) ) ;
#55244=CARTESIAN_POINT ( 'NONE',  ( -5.299128797975815708, -282.0669317393888491, -201.2256419900265598 ) ) ;
#55245=CARTESIAN_POINT ( 'NONE',  ( 37.49873848970126744, -282.6666377438206155, -254.4174803007550167 ) ) ;
#55246=CARTESIAN_POINT ( 'NONE',  ( 23.68369767749559429, -280.8289655848830080, -230.2087408335016505 ) ) ;
#55247=CARTESIAN_POINT ( 'NONE',  ( -31.20066297429009339, -276.1298694293079734, -195.5999559729321220 ) ) ;
#55248=CARTESIAN_POINT ( 'NONE',  ( -24.90781296383362431, -294.8978862385354205, -346.4046464121967119 ) ) ;
#55249=CARTESIAN_POINT ( 'NONE',  ( -95.39914207738490859, -287.9233282611938876, -317.2778553081587916 ) ) ;
#55250=AXIS2_PLACEMENT_3D ( 'NONE', #89927, #76208, #48239 ) ;
#55251=CARTESIAN_POINT ( 'NONE',  ( -107.5719997283207903, -271.6300053544314324, -248.8602684521627282 ) ) ;
#55253=VERTEX_POINT ( 'NONE', #55596 ) ;
#55254=CARTESIAN_POINT ( 'NONE',  ( -90.71201026400952117, -287.2088148994744756, -218.3937290401748328 ) ) ;
#55255=CARTESIAN_POINT ( 'NONE',  ( 30.63473698249595500, -295.0917375002918561, -305.8674062517867469 ) ) ;
#55256=CARTESIAN_POINT ( 'NONE',  ( -1.194397296101256334, -283.2102950782972925, -333.9005952094517511 ) ) ;
#55257=CARTESIAN_POINT ( 'NONE',  ( -39.96694815735507689, -276.1431006282817862, -347.0939478457625569 ) ) ;
#55258=CARTESIAN_POINT ( 'NONE',  ( -81.87810640496687142, -292.1141240881958083, -207.6728311799460016 ) ) ;
#55259=CARTESIAN_POINT ( 'NONE',  ( -89.02603870617329562, -283.4748625758033995, -214.8909160566551293 ) ) ;
#55260=CARTESIAN_POINT ( 'NONE',  ( -7.202393667223206286, -292.7700831896556792, -199.5134292724765430 ) ) ;
#55261=CARTESIAN_POINT ( 'NONE',  ( -61.25793261280417568, -289.7047503125992307, -339.3546054323115868 ) ) ;
#55264=CARTESIAN_POINT ( 'NONE',  ( 167.8059441758928472, 229.7153237395507972, -189.9420329269269416 ) ) ;
#55265=CARTESIAN_POINT ( 'NONE',  ( -37.29506492478459023, -284.5716569555509068, -346.6807208086726177 ) ) ;
#55266=CARTESIAN_POINT ( 'NONE',  ( -37.30987171927208834, -289.5523547857347353, -195.3611179825600175 ) ) ;
#55268=CARTESIAN_POINT ( 'NONE',  ( 32.27446765197596790, -280.1668841413159612, -247.2267995581915727 ) ) ;
#55269=CARTESIAN_POINT ( 'NONE',  ( 38.16080181485249057, -275.4065684828328244, -285.3650005456399867 ) ) ;
#55270=CARTESIAN_POINT ( 'NONE',  ( -54.94823617926331849, -281.8255670592818660, -197.5749555423474533 ) ) ;
#55271=CARTESIAN_POINT ( 'NONE',  ( -81.50230589449645890, -220.2296791547506700, -350.8044924647537073 ) ) ;
#55272=CARTESIAN_POINT ( 'NONE',  ( -6.451800663324420704, -279.0246754427579390, -200.4583245473610020 ) ) ;
#55273=CARTESIAN_POINT ( 'NONE',  ( -111.1280896718952107, -282.4223460673914019, -281.9813032666788217 ) ) ;
#55274=CARTESIAN_POINT ( 'NONE',  ( -48.83908960011165590, -299.6679201047492143, -195.1963459988544400 ) ) ;
#55275=CARTESIAN_POINT ( 'NONE',  ( 35.76960033030849928, -294.0496810488389201, -270.7540019450332807 ) ) ;
#55277=EDGE_LOOP ( 'NONE', ( #17290, #27942, #76646, #49560 ) ) ;
#55278=CARTESIAN_POINT ( 'NONE',  ( -109.1891674642713070, -289.4396237952916522, -254.8955136647435040 ) ) ;
#55279=CARTESIAN_POINT ( 'NONE',  ( 30.45711740953998614, -276.6744201618842567, -306.7590124399724800 ) ) ;
#55280=CARTESIAN_POINT ( 'NONE',  ( 32.86001859858366458, -275.2853248856216055, -250.1625354613445893 ) ) ;
#55281=CARTESIAN_POINT ( 'NONE',  ( -109.8052759601073944, -271.7903385465658062, -245.2509071705767383 ) ) ;
#55286=CARTESIAN_POINT ( 'NONE',  ( -3.466371752806750806, -283.6736478335483298, -335.3881683580153208 ) ) ;
#55287=CARTESIAN_POINT ( 'NONE',  ( 38.60768600563889663, -283.3424564320947070, -272.7411930432493250 ) ) ;
#55288=CARTESIAN_POINT ( 'NONE',  ( -93.50570327252459890, -283.2377208077950854, -317.1531837555374409 ) ) ;
#55289=CARTESIAN_POINT ( 'NONE',  ( 3.388257622749063724, -273.0092043281540555, -208.7572761759778643 ) ) ;
#55290=CARTESIAN_POINT ( 'NONE',  ( 10.04713895627643439, -282.5733485460163479, -213.1525185080326708 ) ) ;
#55291=CARTESIAN_POINT ( 'NONE',  ( 33.55967941179866898, -274.2957006032791583, -290.4995933792133656 ) ) ;
#55293=CARTESIAN_POINT ( 'NONE',  ( -11.39362029786622799, -275.4778510705780263, -201.7435684218430936 ) ) ;
#55296=CARTESIAN_POINT ( 'NONE',  ( -97.57669682175375669, -279.9946897548765037, -222.6546824133990015 ) ) ;
#55300=CARTESIAN_POINT ( 'NONE',  ( -70.54661140398212638, -287.4794191280940936, -202.2601682680719364 ) ) ;
#55301=CARTESIAN_POINT ( 'NONE',  ( -31.59985972116005470, -294.1751196669293904, -343.3471563650673488 ) ) ;
#55302=CARTESIAN_POINT ( 'NONE',  ( -91.53259236698066559, -289.1475959591082301, -324.9948077552997461 ) ) ;
#55303=CARTESIAN_POINT ( 'NONE',  ( 18.55601828459433378, -285.1099397020633432, -221.8490669909610062 ) ) ;
#55304=CARTESIAN_POINT ( 'NONE',  ( 33.24023254658363413, -285.8530342012565484, -249.4943870940143142 ) ) ;
#55305=CARTESIAN_POINT ( 'NONE',  ( -111.3809146095826890, -288.8173498665217949, -268.4130287025081429 ) ) ;
#55306=CARTESIAN_POINT ( 'NONE',  ( -108.4169941214110082, -285.9976925225175819, -252.0462854792802716 ) ) ;
#55307=CARTESIAN_POINT ( 'NONE',  ( 24.40541982995617687, -274.1300837368632415, -313.0220095974415813 ) ) ;
#55308=CARTESIAN_POINT ( 'NONE',  ( 36.94434838036111302, -285.7368933597451814, -253.3318863082909616 ) ) ;
#55309=CARTESIAN_POINT ( 'NONE',  ( -30.73134238605511115, -300.1350572960299132, -195.3588556004923760 ) ) ;
#55310=CARTESIAN_POINT ( 'NONE',  ( 8.708165461508302840, -284.6815505871022083, -210.9520420542893930 ) ) ;
#55312=CARTESIAN_POINT ( 'NONE',  ( 23.87263430292015798, -281.9367189436453032, -230.0675252828383748 ) ) ;
#55313=CARTESIAN_POINT ( 'NONE',  ( 4.557036507022792726, -290.4882716850171960, -332.7672418238798286 ) ) ;
#55317=CARTESIAN_POINT ( 'NONE',  ( -19.60119479712524537, -296.7460420116595401, -343.8628447275620488 ) ) ;
#55319=CARTESIAN_POINT ( 'NONE',  ( -92.75787182491727378, -277.2574126697149381, -219.8235224304492306 ) ) ;
#55320=CARTESIAN_POINT ( 'NONE',  ( -4.663514487870281222, -291.6689447383485572, -200.8176423392138190 ) ) ;
#55321=CARTESIAN_POINT ( 'NONE',  ( -106.7464311612196326, -294.6196705321012246, -295.5998168102003092 ) ) ;
#55322=CARTESIAN_POINT ( 'NONE',  ( 34.71086766197497298, -280.4275378467136193, -284.9043988270296950 ) ) ;
#55323=CARTESIAN_POINT ( 'NONE',  ( 20.12582473539187333, -272.9744513515419726, -223.0451821115256905 ) ) ;
#55324=CARTESIAN_POINT ( 'NONE',  ( 2.493830814584487854, -293.9132260496983804, -208.5402229044700846 ) ) ;
#55325=CARTESIAN_POINT ( 'NONE',  ( -37.37352853689063892, -294.5519495502701943, -195.3611179825600175 ) ) ;
#55326=CARTESIAN_POINT ( 'NONE',  ( -105.3486530527257798, -294.5810064334737604, -305.0862719101137372 ) ) ;
#55327=CARTESIAN_POINT ( 'NONE',  ( 24.05411970751454831, -292.3944528033189840, -315.1549753035525896 ) ) ;
#55328=CARTESIAN_POINT ( 'NONE',  ( -95.40435885385358006, -291.3452768561692210, -315.5932223192789365 ) ) ;
#55330=CARTESIAN_POINT ( 'NONE',  ( -104.8560228691733869, -291.7338019572545136, -242.0438180668773498 ) ) ;
#55332=CARTESIAN_POINT ( 'NONE',  ( 5.958818695645231145, -280.4886725278546464, -332.0972052273217514 ) ) ;
#55333=CARTESIAN_POINT ( 'NONE',  ( 16.73817998885948199, -292.8488599158071111, -221.2526383744979341 ) ) ;
#55334=CARTESIAN_POINT ( 'NONE',  ( 21.06610096577867353, -280.8747130857748857, -220.1660874738981875 ) ) ;
#55335=CARTESIAN_POINT ( 'NONE',  ( -61.22914353509621321, -283.0206303925972406, -343.5955716834060922 ) ) ;
#55336=CARTESIAN_POINT ( 'NONE',  ( 19.19427307647419312, -286.2343163782348938, -319.4663365697116433 ) ) ;
#55337=CARTESIAN_POINT ( 'NONE',  ( -96.10855236157496506, -282.0635665716423546, -315.7395940009587321 ) ) ;
#55338=CARTESIAN_POINT ( 'NONE',  ( 27.27464862055146355, -279.4946470173169359, -229.6734459171293850 ) ) ;
#55339=CARTESIAN_POINT ( 'NONE',  ( 18.13742591029376072, -285.7448594641809336, -217.3358698804441929 ) ) ;
#55341=CARTESIAN_POINT ( 'NONE',  ( 19.95413491869341271, -294.5010696573632458, -223.8263267928029734 ) ) ;
#55342=CARTESIAN_POINT ( 'NONE',  ( -72.55288886850765095, -278.9342408450827406, -338.1900018433767627 ) ) ;
#55343=CARTESIAN_POINT ( 'NONE',  ( -74.02756898543130148, -277.2208424048024540, -333.4977516667271402 ) ) ;
#55344=CARTESIAN_POINT ( 'NONE',  ( -94.71272277688144925, -291.4154704905947710, -219.0038812505702026 ) ) ;
#55345=CARTESIAN_POINT ( 'NONE',  ( -58.11478627734786073, -281.3982086140009073, -343.0640047461504309 ) ) ;
#55346=CARTESIAN_POINT ( 'NONE',  ( 25.05460489774092991, -292.0829286742416571, -231.9228130497185987 ) ) ;
#55347=CARTESIAN_POINT ( 'NONE',  ( -109.6701956138007858, -294.2968592608739300, -290.2002054543653458 ) ) ;
#55350=CARTESIAN_POINT ( 'NONE',  ( 29.54387913903637397, -293.4549884766422565, -299.7602289822567059 ) ) ;
#55352=CARTESIAN_POINT ( 'NONE',  ( 30.89617123739170168, -291.2666405000203440, -285.9686137636504668 ) ) ;
#55353=CARTESIAN_POINT ( 'NONE',  ( -107.9251138741139897, -272.1384861262200729, -239.8598332598646152 ) ) ;
#55354=CARTESIAN_POINT ( 'NONE',  ( 21.92416627033979992, -279.0493296385649842, -223.1402444176585789 ) ) ;
#55355=CARTESIAN_POINT ( 'NONE',  ( -23.88918542111262866, -287.5355938107643965, -194.9923905869694920 ) ) ;
#55356=CARTESIAN_POINT ( 'NONE',  ( -8.252996814476444953, -286.2773262934074410, -203.4070490691913449 ) ) ;
#55357=CARTESIAN_POINT ( 'NONE',  ( -99.75206561250479353, -279.5350699662603802, -309.6438209995825446 ) ) ;
#55358=CARTESIAN_POINT ( 'NONE',  ( -96.93231070470670829, -293.9544938519271113, -315.3355578255349769 ) ) ;
#55359=CARTESIAN_POINT ( 'NONE',  ( -92.93723497903441455, -297.6243472131266117, -319.2191830237677550 ) ) ;
#55360=CARTESIAN_POINT ( 'NONE',  ( -107.9964031095898918, -277.6089295595630801, -250.4388713354596803 ) ) ;
#55362=CARTESIAN_POINT ( 'NONE',  ( -36.89275367695309171, -297.7243499385728569, -193.3822863192873456 ) ) ;
#55363=CARTESIAN_POINT ( 'NONE',  ( -110.5916268880976503, -292.3008018687873459, -283.6186603410305338 ) ) ;
#55364=CARTESIAN_POINT ( 'NONE',  ( 17.00541833075179809, -295.8938911368153413, -323.8480890900463010 ) ) ;
#55366=CARTESIAN_POINT ( 'NONE',  ( -18.43915824921367985, -289.4536710904361598, -341.0295460219195434 ) ) ;
#55368=CARTESIAN_POINT ( 'NONE',  ( 36.96103337391910060, -280.8530205513092142, -289.6464493976515087 ) ) ;
#55369=CARTESIAN_POINT ( 'NONE',  ( -102.2348291789772929, -297.7450393017512624, -229.1034570158358861 ) ) ;
#55370=CARTESIAN_POINT ( 'NONE',  ( -78.89682229393353907, -289.6384780114020145, -206.9464056147878921 ) ) ;
#55371=CARTESIAN_POINT ( 'NONE',  ( -60.14587605445937868, -298.0978450219084834, -196.7820501921080165 ) ) ;
#55375=CARTESIAN_POINT ( 'NONE',  ( -62.51647696985671132, -290.8938532166030200, -342.4512751567758642 ) ) ;
#55376=CARTESIAN_POINT ( 'NONE',  ( -88.52914483777347243, -281.9090924074130839, -206.2264541496106460 ) ) ;
#55377=CARTESIAN_POINT ( 'NONE',  ( 22.80078898073362481, -280.2581365725688443, -222.4215643263058553 ) ) ;
#55378=CARTESIAN_POINT ( 'NONE',  ( -98.07732992441323461, -287.1488889442275081, -226.6218406911590648 ) ) ;
#55379=CARTESIAN_POINT ( 'NONE',  ( 26.65425886802522371, -285.5741825527417177, -228.6103871548034476 ) ) ;
#55380=CARTESIAN_POINT ( 'NONE',  ( -72.75333861237710664, -271.5822585228652883, -204.3788530085386412 ) ) ;
#55381=CARTESIAN_POINT ( 'NONE',  ( -75.02300922096350178, -275.4666289778325563, -206.1030072348783051 ) ) ;
#55382=CARTESIAN_POINT ( 'NONE',  ( -111.2216220126953345, -288.5140864063913568, -279.4754659901390141 ) ) ;
#55383=CARTESIAN_POINT ( 'NONE',  ( -112.0230213362468987, -280.5748415217224760, -257.5937476853273438 ) ) ;
#55386=CARTESIAN_POINT ( 'NONE',  ( 21.32897384886098990, -280.9428830652790907, -226.9033205156976010 ) ) ;
#55387=CARTESIAN_POINT ( 'NONE',  ( 22.20133182572669384, -280.3091536364263447, -227.9521564990508864 ) ) ;
#55388=CARTESIAN_POINT ( 'NONE',  ( -7.990171337955164432, -277.7562238104093240, -341.2271656127474557 ) ) ;
#55389=CARTESIAN_POINT ( 'NONE',  ( -22.62733913665131880, -279.0312568105371156, -195.1307060878413324 ) ) ;
#55390=CARTESIAN_POINT ( 'NONE',  ( 177.9932344209848623, 252.8631895712235576, -164.8680862452318934 ) ) ;
#55391=CARTESIAN_POINT ( 'NONE',  ( 39.31859167701078661, -276.4317044675041757, -265.4428702740854078 ) ) ;
#55392=CARTESIAN_POINT ( 'NONE',  ( -35.86075138741976787, -299.4956160365115352, -193.9499916391053773 ) ) ;
#55395=CARTESIAN_POINT ( 'NONE',  ( 1.486910614065003466, -289.5994750476927493, -332.5428280042053757 ) ) ;
#55396=CARTESIAN_POINT ( 'NONE',  ( 15.99091625240357395, -290.0692590247060139, -324.5601440855464830 ) ) ;
#55397=CARTESIAN_POINT ( 'NONE',  ( -101.7368629529239428, -289.4282941926513786, -305.0684018471576451 ) ) ;
#55398=CARTESIAN_POINT ( 'NONE',  ( -83.23414282389853724, -284.9502863602965022, -208.5418669721679521 ) ) ;
#55399=CARTESIAN_POINT ( 'NONE',  ( 6.793877929583397979, -58.98313164763600724, -354.7002343187792803 ) ) ;
#55400=CARTESIAN_POINT ( 'NONE',  ( -3.269961521395382764, -280.9942813555045404, -335.8394410721698478 ) ) ;
#55401=CARTESIAN_POINT ( 'NONE',  ( 32.12216389915990078, -289.0672458292703482, -244.0314622169746315 ) ) ;
#55402=CARTESIAN_POINT ( 'NONE',  ( -71.74959689872466129, -281.9954652854672190, -335.5286282438998455 ) ) ;
#55403=CARTESIAN_POINT ( 'NONE',  ( -107.5830224914130753, -279.5808595420816687, -292.1508377993539511 ) ) ;
#55404=CARTESIAN_POINT ( 'NONE',  ( -91.00879535272413534, -278.3323750928786353, -320.0112203473791510 ) ) ;
#55405=CARTESIAN_POINT ( 'NONE',  ( -98.72023481205707185, -288.7339307275170199, -316.2160364199178844 ) ) ;
#55406=CARTESIAN_POINT ( 'NONE',  ( -110.0685433276176042, -285.0418659927611316, -295.1596078263626737 ) ) ;
#55407=CARTESIAN_POINT ( 'NONE',  ( -109.2432041649214085, -284.6959570722593753, -297.8902037638685556 ) ) ;
#55408=CARTESIAN_POINT ( 'NONE',  ( 32.96001963823315606, -281.9787327190362021, -290.0249986376510947 ) ) ;
#55411=CARTESIAN_POINT ( 'NONE',  ( -111.6517927650008914, -292.2239280562962449, -285.2022837483743274 ) ) ;
#55412=CARTESIAN_POINT ( 'NONE',  ( -94.33269609112210219, -289.9338557518891548, -219.3187370387785791 ) ) ;
#55413=CARTESIAN_POINT ( 'NONE',  ( 34.85964460119316755, -274.4486703780240759, -258.0238429230757333 ) ) ;
#55415=CARTESIAN_POINT ( 'NONE',  ( -61.56733123551180853, -294.7072671766154599, -343.3991914521322997 ) ) ;
#55416=CARTESIAN_POINT ( 'NONE',  ( -68.07283883817619596, -290.1210344938378398, -203.3673712090817105 ) ) ;
#55417=CARTESIAN_POINT ( 'NONE',  ( -56.08122799540302594, -293.5365395150099062, -342.0159378641242256 ) ) ;
#55418=CARTESIAN_POINT ( 'NONE',  ( -23.69638451457892003, -290.0791089596519328, -342.5306143589440921 ) ) ;
#55419=CARTESIAN_POINT ( 'NONE',  ( -110.9666534002643488, -292.7367265566448395, -255.9984047818169586 ) ) ;
#55420=CARTESIAN_POINT ( 'NONE',  ( 19.02128324634172074, -290.8620007670184577, -220.6099585487555714 ) ) ;
#55421=CARTESIAN_POINT ( 'NONE',  ( -70.20133459584216951, -297.4852658003967463, -337.7935247217671417 ) ) ;
#55422=CARTESIAN_POINT ( 'NONE',  ( -83.80637592691429916, -286.3375077704160390, -213.6874246577449981 ) ) ;
#55423=CARTESIAN_POINT ( 'NONE',  ( -52.88466988958912651, -297.2509308156264751, -343.9564859629384159 ) ) ;
#55424=CARTESIAN_POINT ( 'NONE',  ( -21.72089202138068131, -276.2313206908625602, -196.6427542333496206 ) ) ;
#55425=CARTESIAN_POINT ( 'NONE',  ( -68.10340025477833592, -296.8556995106122258, -199.8922526633819814 ) ) ;
#55426=CARTESIAN_POINT ( 'NONE',  ( 30.06808866905312527, -274.1982649241995205, -300.9208036039907483 ) ) ;
#55427=CARTESIAN_POINT ( 'NONE',  ( 16.31396394556751872, -278.9007586467985220, -218.6891601031146877 ) ) ;
#55428=CARTESIAN_POINT ( 'NONE',  ( 9.305168264481828544, -299.9632585043001995, -196.8572638878959538 ) ) ;
#55429=CARTESIAN_POINT ( 'NONE',  ( 33.17682165268007566, -273.7482668069132501, -240.8008472706179930 ) ) ;
#55431=CARTESIAN_POINT ( 'NONE',  ( -109.4585590065431688, -297.7849363789778749, -285.0707624594489289 ) ) ;
#55433=CARTESIAN_POINT ( 'NONE',  ( -107.9942599148068609, -297.6058988385121893, -251.3176196582970192 ) ) ;
#55435=CARTESIAN_POINT ( 'NONE',  ( 28.90443694933325602, -286.0482791524841559, -306.3847482653974339 ) ) ;
#55436=CARTESIAN_POINT ( 'NONE',  ( -55.29366199708200469, -297.8148464622946676, -199.5505777150535494 ) ) ;
#55437=CARTESIAN_POINT ( 'NONE',  ( -26.62110565877075530, -286.1848046337939877, -194.0575773621118287 ) ) ;
#55438=CARTESIAN_POINT ( 'NONE',  ( -1.814256152264956734, -288.2611825443088378, -338.6512711244930074 ) ) ;
#55439=CARTESIAN_POINT ( 'NONE',  ( -100.1920628284645289, -299.0910493277199294, -228.7655196365475376 ) ) ;
#55440=CARTESIAN_POINT ( 'NONE',  ( 36.64678441054144287, -291.7006130137693276, -281.9104802602840323 ) ) ;
#55441=CARTESIAN_POINT ( 'NONE',  ( 39.02349030844789013, -280.6367521027814860, -261.3790149900602842 ) ) ;
#55443=CARTESIAN_POINT ( 'NONE',  ( -107.9032732156323533, -276.2207428459387302, -295.9286849696143236 ) ) ;
#55445=CARTESIAN_POINT ( 'NONE',  ( -31.85691627504873225, -287.7764633198391948, -343.6038714961763390 ) ) ;
#55448=CARTESIAN_POINT ( 'NONE',  ( -23.43874908825920755, -286.8743885594022913, -344.1143560153843168 ) ) ;
#55449=CARTESIAN_POINT ( 'NONE',  ( -90.63755955995070224, -298.8816266153137917, -219.2390458299260558 ) ) ;
#55450=CARTESIAN_POINT ( 'NONE',  ( -1.891271080300872987, -284.0171449996391857, -338.0506546526542024 ) ) ;
#55451=CARTESIAN_POINT ( 'NONE',  ( -101.4834919000621198, -271.1644893416909667, -230.4218547814903957 ) ) ;
#55452=CARTESIAN_POINT ( 'NONE',  ( 24.13044094101882564, -282.0979335365723273, -309.8263178026162450 ) ) ;
#55453=CARTESIAN_POINT ( 'NONE',  ( -72.20275711917136618, -275.0071378488802907, -205.4962965694338664 ) ) ;
#55454=CARTESIAN_POINT ( 'NONE',  ( -9.624544997989836759, -282.4144454984723325, -200.6706598049773334 ) ) ;
#55455=CARTESIAN_POINT ( 'NONE',  ( -89.45227716404559715, -272.2167422993282457, -218.7984004980284567 ) ) ;
#55457=CARTESIAN_POINT ( 'NONE',  ( 204.8711143770183014, 294.6098302808098879, -54.00000000003475265 ) ) ;
#55458=CARTESIAN_POINT ( 'NONE',  ( -69.50601791590636935, -287.6066210947611808, -202.9875059202372540 ) ) ;
#55460=CARTESIAN_POINT ( 'NONE',  ( 44.71564893372296723, -273.0523547857346784, -270.3937649182068412 ) ) ;
#55462=CARTESIAN_POINT ( 'NONE',  ( -71.50825514478027856, -276.6891662247812178, -339.1855710464828348 ) ) ;
#55463=CARTESIAN_POINT ( 'NONE',  ( -75.28321270252008901, -287.9490731754092394, -336.4435062504490475 ) ) ;
#55464=CARTESIAN_POINT ( 'NONE',  ( -66.81929725816203813, -284.9656697739501965, -337.9157592584721783 ) ) ;
#55465=( BOUNDED_CURVE ( )  B_SPLINE_CURVE ( 2, ( #82439, #11405, #41677, #35544, #63507, #42139, #43102, #86170, #21321, #85250, #18, #35056, #91866, #85711, #48310, #84761, #20397, #93283, #28896, #56387, #27979, #42615, #34131, #84294, #71533, #77211, #63035, #34597, #12339, #41186, #19444, #56869, #5262, #92335, #77688, #14244, #70125, #5722, #27020, #13767, #49727, #6189, #6666, #55909, #63975, #50192, #19911, #27490, #79094, #35996, #78163, #71057, #48782, #78624, #64457, #28435, #12839, #70595, #72009, #57328, #7126, #49268, #20856, #64915, #13301, #92816, #65372, #66286, #952, #29830, #50675, #23648, #1399, #80463, #58713, #65844, #86633, #22703, #8952, #87557, #51128, #30286, #15151, #43557, #72453, #51577, #21801, #59173, #79561, #37832, #88018, #15611, #29370, #14704, #483, #44483, #72909, #8498, #36457, #8034, #22255, #74292, #58262, #23173, #16084, #36930, #73388, #37376, #52056, #80939, #44937, #80011, #73838, #9416, #66738, #1864, #87105, #38302, #30755, #44011, #59657, #88501, #67217 ),
 .UNSPECIFIED., .F., .F. ) 
 B_SPLINE_CURVE_WITH_KNOTS ( ( 3, 2, 2, 2, 2, 2, 2, 2, 2, 2, 2, 2, 2, 2, 2, 2, 2, 2, 2, 2, 2, 2, 2, 2, 2, 2, 2, 2, 2, 2, 2, 2, 2, 2, 2, 2, 2, 2, 2, 2, 2, 2, 2, 2, 2, 2, 2, 2, 2, 2, 2, 2, 2, 2, 2, 2, 2, 2, 2, 2, 2, 3 ),
 ( -0.05135551144988961814, 0.000000000000000000, 0.01428571428571429047, 0.02857142857142856707, 0.04285714285714285754, 0.05714285714285713413, 0.07142857142857142461, 0.08571428571428571508, 0.09999999999999997780, 0.1142857142857142960, 0.1285714285714285587, 0.1428571428571428492, 0.1571428571428571397, 0.1714285714285714302, 0.1857142857142857206, 0.2000000000000000389, 0.2142857142857142738, 0.2285714285714285643, 0.2428571428571429103, 0.2571428571428571175, 0.2714285714285714635, 0.2857142857142856984, 0.3000000000000000444, 0.3142857142857142794, 0.3285714285714286254, 0.3428571428571428603, 0.3571428571428572063, 0.3714285714285714413, 0.3857142857142857872, 0.4000000000000000222, 0.4142857142857143682, 0.4285714285714286031, 0.4428571428571428381, 0.4571428571428571841, 0.4714285714285714191, 0.4857142857142857650, 0.5000000000000000000, 0.5142857142857142350, 0.5285714285714285809, 0.5428571428571428159, 0.5571428571428571619, 0.5714285714285713969, 0.5857142857142857428, 0.5999999999999999778, 0.6142857142857143238, 0.6285714285714285587, 0.6428571428571429047, 0.6571428571428571397, 0.6714285714285713746, 0.6857142857142857206, 0.6999999999999999556, 0.7142857142857143016, 0.7285714285714285365, 0.7428571428571428825, 0.7571428571428571175, 0.7714285714285714635, 0.7857142857142856984, 0.8000000000000000444, 0.8142857142857142794, 0.8285714285714287364, 0.8428571428571428603, 0.8500000000000000888 ),
 .UNSPECIFIED. ) 
 CURVE ( )  GEOMETRIC_REPRESENTATION_ITEM ( )  RATIONAL_B_SPLINE_CURVE ( ( 1.000000000000000000, 1.000000000000000000, 1.000000000000000000, 0.9749279121818236193, 1.000000000000000000, 0.9749279121818236193, 1.000000000000000000, 0.9749279121818236193, 1.000000000000000000, 0.9749279121818236193, 1.000000000000000000, 0.9749279121818236193, 1.000000000000000000, 0.9749279121818236193, 1.000000000000000000, 0.9749279121818236193, 1.000000000000000000, 0.9749279121818236193, 1.000000000000000000, 0.9749279121818236193, 1.000000000000000000, 0.9749279121818236193, 1.000000000000000000, 0.9749279121818236193, 1.000000000000000000, 0.9749279121818236193, 1.000000000000000000, 0.9749279121818236193, 1.000000000000000000, 0.9749279121818236193, 1.000000000000000000, 0.9749279121818236193, 1.000000000000000000, 0.9749279121818236193, 1.000000000000000000, 0.9749279121818236193, 1.000000000000000000, 0.9749279121818236193, 1.000000000000000000, 0.9749279121818236193, 1.000000000000000000, 0.9749279121818236193, 1.000000000000000000, 0.9749279121818236193, 1.000000000000000000, 0.9749279121818236193, 1.000000000000000000, 0.9749279121818236193, 1.000000000000000000, 0.9749279121818236193, 1.000000000000000000, 0.9749279121818236193, 1.000000000000000000, 0.9749279121818236193, 1.000000000000000000, 0.9749279121818236193, 1.000000000000000000, 0.9749279121818236193, 1.000000000000000000, 0.9749279121818236193, 1.000000000000000000, 0.9749279121818236193, 1.000000000000000000, 0.9749279121818236193, 1.000000000000000000, 0.9749279121818236193, 1.000000000000000000, 0.9749279121818236193, 1.000000000000000000, 0.9749279121818236193, 1.000000000000000000, 0.9749279121818236193, 1.000000000000000000, 0.9749279121818236193, 1.000000000000000000, 0.9749279121818236193, 1.000000000000000000, 0.9749279121818236193, 1.000000000000000000, 0.9749279121818236193, 1.000000000000000000, 0.9749279121818236193, 1.000000000000000000, 0.9749279121818236193, 1.000000000000000000, 0.9749279121818236193, 1.000000000000000000, 0.9749279121818236193, 1.000000000000000000, 0.9749279121818236193, 1.000000000000000000, 0.9749279121818236193, 1.000000000000000000, 0.9749279121818236193, 1.000000000000000000, 0.9749279121818236193, 1.000000000000000000, 0.9749279121818236193, 1.000000000000000000, 0.9749279121818236193, 1.000000000000000000, 0.9749279121818236193, 1.000000000000000000, 0.9749279121818236193, 1.000000000000000000, 0.9749279121818236193, 1.000000000000000000, 0.9749279121818236193, 1.000000000000000000, 0.9749279121818236193, 1.000000000000000000, 0.9749279121818236193, 1.000000000000000000, 0.9749279121818236193, 1.000000000000000000, 0.9749279121818236193, 1.000000000000000000, 0.9749279121818236193, 1.000000000000000000, 0.9749279121818236193, 1.000000000000000000, 0.9874639560909115321, 0.9874639560909117542 ) ) 
 REPRESENTATION_ITEM ( '' )  );
#55466=CARTESIAN_POINT ( 'NONE',  ( 3.594608448287563096, -278.0913826659201504, -331.7668103410704816 ) ) ;
#55467=CARTESIAN_POINT ( 'NONE',  ( -107.6775978405456016, -285.5928995964299588, -300.3538581988019587 ) ) ;
#55468=CARTESIAN_POINT ( 'NONE',  ( -10.84667839444351856, -281.4938731697979506, -338.8630986575993802 ) ) ;
#55469=CARTESIAN_POINT ( 'NONE',  ( 18.53634522016949404, -282.8556198287805046, -220.3346779906016764 ) ) ;
#55470=CARTESIAN_POINT ( 'NONE',  ( -35.52591442282115963, -274.2409939280164508, -193.3694003170991209 ) ) ;
#55471=CARTESIAN_POINT ( 'NONE',  ( -11.86818737651423916, -276.5629683692066578, -343.0813416925631145 ) ) ;
#55473=CARTESIAN_POINT ( 'NONE',  ( -102.7205993646781934, -297.9958500886361890, -305.9548495919689799 ) ) ;
#55476=CARTESIAN_POINT ( 'NONE',  ( -107.7320901837979932, -295.0546827823979470, -242.1934993061658190 ) ) ;
#55477=CARTESIAN_POINT ( 'NONE',  ( 34.43512935225187022, -274.8800081481237498, -256.7201799077768669 ) ) ;
#55478=CARTESIAN_POINT ( 'NONE',  ( -14.93625191785613460, -299.4061590513995839, -193.6662267349441890 ) ) ;
#55479=CARTESIAN_POINT ( 'NONE',  ( 31.91498412446033939, -288.9669872684551706, -244.1112805909705230 ) ) ;
#55480=CARTESIAN_POINT ( 'NONE',  ( 25.94760616720495960, -295.6389878986219060, -312.9894121227993082 ) ) ;
#55481=CARTESIAN_POINT ( 'NONE',  ( 26.19104245480922444, -295.3239925013591005, -313.1583064233602158 ) ) ;
#55482=CARTESIAN_POINT ( 'NONE',  ( -101.8722935725086955, -292.0435366293702373, -308.3554825400511845 ) ) ;
#55483=CARTESIAN_POINT ( 'NONE',  ( -3.496160583036511671, -278.4997593273849930, -203.6047763549147760 ) ) ;
#55484=CARTESIAN_POINT ( 'NONE',  ( -106.8678382121186416, -280.8223266964639038, -243.6190552837798293 ) ) ;
#55485=CARTESIAN_POINT ( 'NONE',  ( -76.43470201132666375, -293.6588031990233389, -333.7698735089981028 ) ) ;
#55486=CARTESIAN_POINT ( 'NONE',  ( -27.50855455054090726, -284.7890556680354166, -345.5376198938438392 ) ) ;
#55487=CARTESIAN_POINT ( 'NONE',  ( -106.8208824783783228, -283.7836976823479063, -246.8170190287729895 ) ) ;
#55488=CARTESIAN_POINT ( 'NONE',  ( 66.71607493782951792, 46.51903866668713761, -318.0724619622529872 ) ) ;
#55490=CARTESIAN_POINT ( 'NONE',  ( -73.56243245377845597, -285.2240150428240213, -206.9419965642647412 ) ) ;
#55493=CARTESIAN_POINT ( 'NONE',  ( 13.48624932932764153, -283.4401334733751128, -327.8601380250025841 ) ) ;
#55494=CARTESIAN_POINT ( 'NONE',  ( -35.39401571080843922, -274.4105157603730731, -197.3534446868073360 ) ) ;
#55495=CARTESIAN_POINT ( 'NONE',  ( -65.71594498117595151, -284.4841220575337388, -199.1929026543034524 ) ) ;
#55496=CARTESIAN_POINT ( 'NONE',  ( -41.00918210546713993, -280.9483383741807643, -193.6709142031657223 ) ) ;
#55498=CARTESIAN_POINT ( 'NONE',  ( -14.77608751163456624, -278.2852054993145430, -343.3102098040038754 ) ) ;
#55499=CARTESIAN_POINT ( 'NONE',  ( -45.27112193987900923, -280.6057585057944266, -193.8200478499758219 ) ) ;
#55500=CARTESIAN_POINT ( 'NONE',  ( 7.450504543161054372, -278.1952119285919025, -214.2458315076590907 ) ) ;
#55501=CARTESIAN_POINT ( 'NONE',  ( 122.6214869821080811, 149.1237144905377932, -263.6315619574343145 ) ) ;
#55503=CARTESIAN_POINT ( 'NONE',  ( 16.75491512059070942, -276.8239737314698345, -218.5794173880239271 ) ) ;
#55504=CARTESIAN_POINT ( 'NONE',  ( 138.3973862054802737, 180.7445933655617978, -241.2771218006182039 ) ) ;
#55505=CARTESIAN_POINT ( 'NONE',  ( -108.7944505226338947, -276.8518797301865106, -248.7659503619966870 ) ) ;
#55506=CARTESIAN_POINT ( 'NONE',  ( 32.38553520393038099, -294.9222933365073800, -240.1603454029673230 ) ) ;
#55507=CARTESIAN_POINT ( 'NONE',  ( -108.0703058816943383, -295.6565544052842824, -288.8864808610924797 ) ) ;
#55508=CARTESIAN_POINT ( 'NONE',  ( -73.39932000544710888, -291.0946126367481952, -202.3802468904231944 ) ) ;
#55510=CARTESIAN_POINT ( 'NONE',  ( -113.0156614526297290, -295.2614842633988701, -259.6808898944332213 ) ) ;
#55511=CARTESIAN_POINT ( 'NONE',  ( 35.06513564341257450, -286.1391030515925422, -284.6983745206543972 ) ) ;
#55512=CARTESIAN_POINT ( 'NONE',  ( 26.87280497923282852, -295.9150488210141248, -307.6084375127143176 ) ) ;
#55513=CARTESIAN_POINT ( 'NONE',  ( -89.23069155448426670, -285.1159819910635633, -322.4784343670461340 ) ) ;
#55515=CARTESIAN_POINT ( 'NONE',  ( -64.31738168574405279, -292.6499734411429472, -198.4362540265437929 ) ) ;
#55516=CARTESIAN_POINT ( 'NONE',  ( 9.953300776215803225, -282.8724606098635945, -326.1158162903707307 ) ) ;
#55517=CARTESIAN_POINT ( 'NONE',  ( -110.8387786517707809, -295.0743203415212861, -291.9988081994144977 ) ) ;
#55518=CARTESIAN_POINT ( 'NONE',  ( -111.4796996524113268, -291.6089736175756002, -250.1191914034936588 ) ) ;
#55519=CARTESIAN_POINT ( 'NONE',  ( -62.73741867947213535, -289.8662440842581987, -343.0437894202646021 ) ) ;
#55520=CARTESIAN_POINT ( 'NONE',  ( 16.01241423388361440, -288.4360963772322748, -320.2581557606845877 ) ) ;
#55523=CARTESIAN_POINT ( 'NONE',  ( -87.76542100751417763, -297.6078110243569768, -326.9801367653643069 ) ) ;
#55524=CARTESIAN_POINT ( 'NONE',  ( -106.0629662370787543, -295.6715756371194175, -236.7354454123922949 ) ) ;
#55525=CARTESIAN_POINT ( 'NONE',  ( 31.29500917669439275, -280.2695869896268164, -244.6732345817005978 ) ) ;
#55528=CARTESIAN_POINT ( 'NONE',  ( 36.52854623391771582, -274.7877249209018373, -248.6641078151613726 ) ) ;
#55529=CARTESIAN_POINT ( 'NONE',  ( -93.25796935765919216, -295.7091383813242942, -222.3408959508808493 ) ) ;
#55530=CARTESIAN_POINT ( 'NONE',  ( -16.00353612843884576, -278.6338251294960742, -341.5174078355344136 ) ) ;
#55531=CARTESIAN_POINT ( 'NONE',  ( -38.07112242273067437, -272.1825007806498320, -196.1294978547597054 ) ) ;
#55532=CARTESIAN_POINT ( 'NONE',  ( -97.50008032437499139, -297.1740657082341386, -312.4098967690163136 ) ) ;
#55533=CARTESIAN_POINT ( 'NONE',  ( -65.70495337640026889, -298.7518997724627070, -202.7611776031480417 ) ) ;
#55535=CARTESIAN_POINT ( 'NONE',  ( -88.05763163336409605, -297.3475653679960828, -327.3030695434280801 ) ) ;
#55536=CARTESIAN_POINT ( 'NONE',  ( -4.388251233285046737, -296.4635845200466520, -195.2056462083211841 ) ) ;
#55537=CARTESIAN_POINT ( 'NONE',  ( -88.00720874947627692, -291.9722842573880257, -217.5948646665382853 ) ) ;
#55538=CARTESIAN_POINT ( 'NONE',  ( -84.19030521499225017, -289.9677289119507577, -213.6109363365657714 ) ) ;
#55540=CARTESIAN_POINT ( 'NONE',  ( 25.27316682631609268, -275.4515324645817600, -225.6294632512385192 ) ) ;
#55541=CARTESIAN_POINT ( 'NONE',  ( -96.90244113493012890, -297.4751434899372953, -228.1165252217108446 ) ) ;
#55542=CARTESIAN_POINT ( 'NONE',  ( 0.5251509340085595001, -282.5336657128820548, -205.1518274706764089 ) ) ;
#55543=CARTESIAN_POINT ( 'NONE',  ( 21.60154766256311731, -279.5771174516640372, -221.5862083013473978 ) ) ;
#55544=CARTESIAN_POINT ( 'NONE',  ( -82.49314110336433714, -276.9996492523249572, -332.6078862854157592 ) ) ;
#55545=CARTESIAN_POINT ( 'NONE',  ( 22.71148703111292377, -281.3304858494317386, -312.1488726383479388 ) ) ;
#55546=CARTESIAN_POINT ( 'NONE',  ( 29.43646660842806995, -280.0076609225698689, -304.8677096843214827 ) ) ;
#55548=CARTESIAN_POINT ( 'NONE',  ( 17.73855798917262305, -273.4344786995096115, -221.4845631202330765 ) ) ;
#55549=CARTESIAN_POINT ( 'NONE',  ( -91.90764182733370546, -281.2742061657593808, -218.8322374065569988 ) ) ;
#55552=CARTESIAN_POINT ( 'NONE',  ( 18.48403035578103015, -296.9817873043560894, -194.3908963028880237 ) ) ;
#55553=CARTESIAN_POINT ( 'NONE',  ( -111.2321641310948763, -290.8238438703999691, -248.7001085550341202 ) ) ;
#55555=CARTESIAN_POINT ( 'NONE',  ( 36.11951409089245146, -277.7570510648502591, -286.3423530635178054 ) ) ;
#55556=CARTESIAN_POINT ( 'NONE',  ( -13.40362284056542563, -272.3628528587607889, -199.2839127544727091 ) ) ;
#55558=CARTESIAN_POINT ( 'NONE',  ( -109.7214204775096533, -286.1943910878828774, -292.0967853559159266 ) ) ;
#55561=CARTESIAN_POINT ( 'NONE',  ( -40.83110399604597518, -287.0958686692045490, -345.2925181388677061 ) ) ;
#55562=CARTESIAN_POINT ( 'NONE',  ( 202.9738562182569694, 293.9636489450776367, -54.00000000000000000 ) ) ;
#55563=CARTESIAN_POINT ( 'NONE',  ( 12.61395769135607736, -293.1322295059306384, -324.2040166919188096 ) ) ;
#55564=CARTESIAN_POINT ( 'NONE',  ( 11.97198968448825873, -284.8853739300199095, -214.8030651670278814 ) ) ;
#55566=CARTESIAN_POINT ( 'NONE',  ( -2.229372256407885722, -292.5872080975239555, -336.6342277833913954 ) ) ;
#55567=CARTESIAN_POINT ( 'NONE',  ( -33.74050798617618341, -284.5765813893596032, -194.1394729668528214 ) ) ;
#55568=CARTESIAN_POINT ( 'NONE',  ( -34.30053951456762462, -281.6911172414450562, -196.6111209455514768 ) ) ;
#55569=CARTESIAN_POINT ( 'NONE',  ( 25.21194345192014552, -288.1687898585081484, -226.1225567101169815 ) ) ;
#55570=CARTESIAN_POINT ( 'NONE',  ( 38.69654786586400519, -279.7869057944955102, -269.9583100898284442 ) ) ;
#55571=CARTESIAN_POINT ( 'NONE',  ( -48.06098284628401274, -289.1921850050840703, -342.6208443211500025 ) ) ;
#55572=CARTESIAN_POINT ( 'NONE',  ( -11.55353154165473661, -281.8198655261309682, -201.3844866885457634 ) ) ;
#55573=CARTESIAN_POINT ( 'NONE',  ( -59.79288494713743063, -280.5567011948643312, -200.6761909063671396 ) ) ;
#55574=CARTESIAN_POINT ( 'NONE',  ( 11.00262234227823299, -288.6968189920589793, -212.4896453108611922 ) ) ;
#55576=CARTESIAN_POINT ( 'NONE',  ( -5.114264152580068057, -274.4647670537403883, -200.4297775803843535 ) ) ;
#55577=CARTESIAN_POINT ( 'NONE',  ( -105.5404452068812304, -292.1310368509668365, -300.8329939880798634 ) ) ;
#55579=CARTESIAN_POINT ( 'NONE',  ( -19.05039376806008633, -297.3376638359844719, -350.3538533559490702 ) ) ;
#55581=CARTESIAN_POINT ( 'NONE',  ( 24.64741721620444181, -272.9770163691381413, -227.8250279221243204 ) ) ;
#55583=CARTESIAN_POINT ( 'NONE',  ( -70.47859530821351370, -293.8815144607628440, -338.9931630804020983 ) ) ;
#55584=CARTESIAN_POINT ( 'NONE',  ( -102.1169269822903090, -272.3625217312203404, -236.3684310538140210 ) ) ;
#55585=CARTESIAN_POINT ( 'NONE',  ( 32.98102004045814795, -289.3635330527375231, -292.5634128866782930 ) ) ;
#55586=CARTESIAN_POINT ( 'NONE',  ( 24.99586053098165905, -283.8577910119429362, -310.3552836523294900 ) ) ;
#55587=CARTESIAN_POINT ( 'NONE',  ( -51.55775109786338817, -290.6558347610954911, -345.4378133426385489 ) ) ;
#55588=CARTESIAN_POINT ( 'NONE',  ( -100.2654114290711505, -291.2888686213889855, -313.8801348498201378 ) ) ;
#55589=CARTESIAN_POINT ( 'NONE',  ( -57.96822921182693023, -287.7860059551414338, -198.1991730765212480 ) ) ;
#55590=CARTESIAN_POINT ( 'NONE',  ( -101.8923791302096191, -279.2712278385557170, -228.2859501127942679 ) ) ;
#55591=CARTESIAN_POINT ( 'NONE',  ( -103.3569439115035209, -294.1451416631172719, -307.2281958411635969 ) ) ;
#55592=CARTESIAN_POINT ( 'NONE',  ( -1.636023932056818397, -282.4254500264314061, -338.5821168898514770 ) ) ;
#55593=CARTESIAN_POINT ( 'NONE',  ( -3.563451093186552843, -276.3632319589444251, -204.2416654072322899 ) ) ;
#55594=CARTESIAN_POINT ( 'NONE',  ( 7.399455738971494334, -283.1948066931273615, -214.2051214447836571 ) ) ;
#55595=CARTESIAN_POINT ( 'NONE',  ( 36.65334540946774666, -273.5723328426788044, -253.0212941062590062 ) ) ;
#55596=CARTESIAN_POINT ( 'NONE',  ( 133.0872704186301405, -299.5541904835127980, -189.2068768330456123 ) ) ;
#55597=CARTESIAN_POINT ( 'NONE',  ( 35.48981690850820314, -281.1441792772546933, -276.7627667117184274 ) ) ;
#55598=CARTESIAN_POINT ( 'NONE',  ( -105.9827270148045386, -279.3165397582349101, -304.4865625263158222 ) ) ;
#55599=CARTESIAN_POINT ( 'NONE',  ( -3.581989427031941897, -285.5455876395546397, -201.4038876781254714 ) ) ;
#55600=CARTESIAN_POINT ( 'NONE',  ( -75.52128544669649557, -293.2959112135206396, -206.8954906990949780 ) ) ;
#55601=CARTESIAN_POINT ( 'NONE',  ( -29.93710617173993427, -275.7445226842622219, -194.5217324153228446 ) ) ;
#55602=CARTESIAN_POINT ( 'NONE',  ( -21.47352411282671980, -275.5667094868534832, -195.5179535560141630 ) ) ;
#55603=CARTESIAN_POINT ( 'NONE',  ( 33.58602562233892286, -275.6139639127588339, -287.6839082804112877 ) ) ;
#55604=CARTESIAN_POINT ( 'NONE',  ( -68.02417613890577286, -297.4560484359759585, -338.6292065791885761 ) ) ;
#55605=CARTESIAN_POINT ( 'NONE',  ( -112.0570084947017477, -282.6168989365954189, -265.3168681408515113 ) ) ;
#55606=CARTESIAN_POINT ( 'NONE',  ( 11.10877385490507407, -292.3684952848250873, -210.4736760558672017 ) ) ;
#55607=CARTESIAN_POINT ( 'NONE',  ( 23.63878784852626680, -272.9843932777092732, -227.2898600109737686 ) ) ;
#55608=CARTESIAN_POINT ( 'NONE',  ( -17.90848375983574314, -290.4057607847047393, -344.0414444956037414 ) ) ;
#55609=CARTESIAN_POINT ( 'NONE',  ( -17.33508574209895059, -291.2366728098951967, -199.7819822093789242 ) ) ;
#55611=CARTESIAN_POINT ( 'NONE',  ( -14.02882395874058830, -290.9233845878376883, -197.5380184614061818 ) ) ;
#55612=CARTESIAN_POINT ( 'NONE',  ( -105.1342552513342952, -289.8541907227410093, -297.6309001967361496 ) ) ;
#55614=CARTESIAN_POINT ( 'NONE',  ( 23.90368209773672703, -289.2489040155889484, -316.5184106539559252 ) ) ;
#55615=CARTESIAN_POINT ( 'NONE',  ( -103.1482246355916033, -278.4559834648771925, -302.1259906924534562 ) ) ;
#55617=CARTESIAN_POINT ( 'NONE',  ( -39.11453006185769965, -293.9942459872765426, -347.0315137352340003 ) ) ;
#55618=CARTESIAN_POINT ( 'NONE',  ( -64.51893673637594873, -286.3579673822758309, -198.4115071107036101 ) ) ;
#55619=CARTESIAN_POINT ( 'NONE',  ( -110.2033003136022131, -284.5723902959645102, -295.1992239871389643 ) ) ;
#55620=CARTESIAN_POINT ( 'NONE',  ( 3.405537827692454833, -282.8211910679626726, -331.0172508417033441 ) ) ;
#55621=CARTESIAN_POINT ( 'NONE',  ( 203.5337727339234846, 295.8836732959281903, -68.67824016207623572 ) ) ;
#55622=CARTESIAN_POINT ( 'NONE',  ( 192.4874460990043303, 278.9581800658359043, -125.3567854953941350 ) ) ;
#55623=CARTESIAN_POINT ( 'NONE',  ( 120.3257472410092106, 148.3080601949953348, -260.4889484542558193 ) ) ;
#55624=CARTESIAN_POINT ( 'NONE',  ( -0.4560453400966971160, -273.7531173004441030, -207.1638205314783931 ) ) ;
#55625=CARTESIAN_POINT ( 'NONE',  ( 35.41109380573036702, -274.5961976119448309, -279.7796281686540283 ) ) ;
#55626=CARTESIAN_POINT ( 'NONE',  ( -106.4552899028562933, -296.4942700314139188, -236.5552218770223760 ) ) ;
#55627=CARTESIAN_POINT ( 'NONE',  ( 122.7515402636430224, 147.2049715914294268, -260.8663683293274289 ) ) ;
#55628=CARTESIAN_POINT ( 'NONE',  ( 14.53640247338804770, -275.0254564862075313, -326.6645220150668933 ) ) ;
#55629=CARTESIAN_POINT ( 'NONE',  ( -110.5888894825546629, -274.4550657320833125, -259.3883154377897995 ) ) ;
#55631=CARTESIAN_POINT ( 'NONE',  ( -54.55409744218442825, -298.7774356042808677, -195.5510010799730480 ) ) ;
#55632=CARTESIAN_POINT ( 'NONE',  ( 5.886078104987047865, -288.9407488534707227, -329.3253402771463243 ) ) ;
#55633=CARTESIAN_POINT ( 'NONE',  ( -36.26643213138716249, -295.8418579235143397, -347.2051944878751897 ) ) ;
#55634=CARTESIAN_POINT ( 'NONE',  ( -111.1545745462997417, -296.7714692090581252, -292.1144043037991764 ) ) ;
#55635=CARTESIAN_POINT ( 'NONE',  ( -25.41118314430918801, -292.3750007293102158, -198.2911504901928481 ) ) ;
#55636=EDGE_LOOP ( 'NONE', ( #6505, #58311, #43291, #68761, #49564 ) ) ;
#55637=CARTESIAN_POINT ( 'NONE',  ( 11.78722809278406736, -278.2960936690671474, -327.7689798758927964 ) ) ;
#55638=CARTESIAN_POINT ( 'NONE',  ( 33.11910213914773493, -280.6654289443937955, -239.4612434371679512 ) ) ;
#55639=CIRCLE ( 'NONE', #7306, 2.395975569037533948 ) ;
#55640=CARTESIAN_POINT ( 'NONE',  ( -9.889073925254171726, -277.6258911462621199, -338.2699548257710944 ) ) ;
#55641=CARTESIAN_POINT ( 'NONE',  ( -8.251561255757351887, -278.4365837355462077, -340.5730644662727400 ) ) ;
#55642=CARTESIAN_POINT ( 'NONE',  ( -45.49721202029022038, -275.1749793123691461, -345.3256222091466157 ) ) ;
#55643=CARTESIAN_POINT ( 'NONE',  ( -84.14645356983561442, -298.0404107818304738, -214.1415903054838736 ) ) ;
#55644=CARTESIAN_POINT ( 'NONE',  ( -106.3521216461459602, -295.4666160159509900, -244.6616095124171864 ) ) ;
#55646=CARTESIAN_POINT ( 'NONE',  ( -71.21315557542598640, -280.1092840815544491, -201.2796341432523093 ) ) ;
#55647=CARTESIAN_POINT ( 'NONE',  ( 15.59934075976178747, -276.4433566139026084, -320.6228946544690643 ) ) ;
#55648=CARTESIAN_POINT ( 'NONE',  ( -57.60906701975474675, -284.4807686903452009, -196.5326051539492767 ) ) ;
#55649=CARTESIAN_POINT ( 'NONE',  ( -69.95714607383332861, -299.6237110336759315, -202.6391782771511600 ) ) ;
#55651=CARTESIAN_POINT ( 'NONE',  ( 17.01743078045893398, -286.0495725490682730, -221.3762336936270287 ) ) ;
#55652=CARTESIAN_POINT ( 'NONE',  ( 11.99778753103542961, -278.9892213532961023, -215.1923861784540861 ) ) ;
#55653=CARTESIAN_POINT ( 'NONE',  ( -41.06297474710797246, -278.5791259067076453, -196.8660362883793198 ) ) ;
#55654=CARTESIAN_POINT ( 'NONE',  ( -43.06760934430345600, -281.2046985372259655, -344.6316517377554192 ) ) ;
#55655=CARTESIAN_POINT ( 'NONE',  ( 23.21259941325403631, -288.9481928874927803, -226.0248794563007380 ) ) ;
#55656=CARTESIAN_POINT ( 'NONE',  ( -108.5536175172389619, -279.5233021261240083, -288.1890860987542169 ) ) ;
#55658=CARTESIAN_POINT ( 'NONE',  ( 3.042594796722233763, -294.5941410503118050, -207.1006052751409356 ) ) ;
#55659=CARTESIAN_POINT ( 'NONE',  ( -74.85569394479161076, -275.7844272069818885, -336.4419342769684818 ) ) ;
#55661=CARTESIAN_POINT ( 'NONE',  ( -26.99890439060824576, -277.5685812009255073, -342.7276796274720709 ) ) ;
#55662=CARTESIAN_POINT ( 'NONE',  ( 36.35327034838019955, -283.7419359996447383, -285.1624610414698964 ) ) ;
#55663=CARTESIAN_POINT ( 'NONE',  ( 83.14890176555634582, -299.5541904835127980, -195.3611179825600175 ) ) ;
#55664=CARTESIAN_POINT ( 'NONE',  ( -48.62927324826024034, -291.1148120146132783, -345.1261981136486838 ) ) ;
#55665=CARTESIAN_POINT ( 'NONE',  ( -98.42176093626626709, -293.9599617903735407, -313.9055724975239627 ) ) ;
#55667=CARTESIAN_POINT ( 'NONE',  ( -64.48057318514403846, -284.9039561673485537, -198.4606790583654004 ) ) ;
#55669=CARTESIAN_POINT ( 'NONE',  ( -76.81508418721976739, -272.1961921824168940, -208.3684133438687525 ) ) ;
#55670=CARTESIAN_POINT ( 'NONE',  ( -33.41988252052209418, -290.2415950093939045, -196.2168772655398925 ) ) ;
#55673=CARTESIAN_POINT ( 'NONE',  ( -34.96246114849688524, -290.5613764734843016, -194.0785186837560445 ) ) ;
#55674=CARTESIAN_POINT ( 'NONE',  ( -18.41250031138758914, -284.5324909898027386, -196.7155727485262560 ) ) ;
#55675=CARTESIAN_POINT ( 'NONE',  ( -73.86370777302514057, -286.9822846621844405, -206.4597448808022477 ) ) ;
#55677=CARTESIAN_POINT ( 'NONE',  ( -19.78698905443609135, -287.0865211982446681, -199.3369400883534865 ) ) ;
#55678=CARTESIAN_POINT ( 'NONE',  ( -19.79478280444287819, -294.2564015011995480, -197.0236909666916176 ) ) ;
#55679=CARTESIAN_POINT ( 'NONE',  ( 23.19895576365909307, -274.2449536268571251, -315.5733197082653305 ) ) ;
#55680=CARTESIAN_POINT ( 'NONE',  ( 36.04375762715931586, -276.1776722089371674, -293.6058782860841347 ) ) ;
#55681=CARTESIAN_POINT ( 'NONE',  ( 10.23148833066985119, -290.7818777374869228, -211.5902411261003522 ) ) ;
#55682=CARTESIAN_POINT ( 'NONE',  ( -62.04762978673585394, -279.7397439990473913, -197.3760363536219984 ) ) ;
#55683=CARTESIAN_POINT ( 'NONE',  ( -48.00359504862603188, -297.1681962995274375, -344.2929853756847365 ) ) ;
#55686=CARTESIAN_POINT ( 'NONE',  ( -83.94776212069248800, -284.0814448168353010, -213.4696746476450926 ) ) ;
#55687=CARTESIAN_POINT ( 'NONE',  ( 31.71421918993832989, -279.9358960430425896, -299.7559121142176650 ) ) ;
#55689=CARTESIAN_POINT ( 'NONE',  ( 38.93829113487036153, -274.0065691618967776, -268.3435244019307220 ) ) ;
#55690=CARTESIAN_POINT ( 'NONE',  ( -64.37854747591299542, -276.7630070288747106, -338.3332230366665954 ) ) ;
#55691=CARTESIAN_POINT ( 'NONE',  ( -18.02025417391305595, -296.3186316492326569, -341.4764431728233376 ) ) ;
#55692=CARTESIAN_POINT ( 'NONE',  ( -28.24795573831202233, -279.0851709983578530, -194.1578794746408505 ) ) ;
#55693=CARTESIAN_POINT ( 'NONE',  ( -93.25429658683719936, -296.8231378173207986, -317.6794842056817174 ) ) ;
#55694=CARTESIAN_POINT ( 'NONE',  ( -109.8728282831767729, -297.5588150344766518, -294.7031335299384978 ) ) ;
#55695=CARTESIAN_POINT ( 'NONE',  ( -86.09871264348110742, -297.1866082164692671, -216.0310734854319037 ) ) ;
#55696=CARTESIAN_POINT ( 'NONE',  ( -111.9653373810833017, -292.6486687494431749, -262.8568918128862606 ) ) ;
#55697=CARTESIAN_POINT ( 'NONE',  ( -76.10855650049418841, -285.7161634103759980, -203.7705439254983162 ) ) ;
#55698=CARTESIAN_POINT ( 'NONE',  ( 38.47115475176315158, -273.7021723269643303, -271.1822867159073098 ) ) ;
#55699=CARTESIAN_POINT ( 'NONE',  ( -71.90837130967148028, -289.3298041366661550, -339.1662431401754816 ) ) ;
#55700=CARTESIAN_POINT ( 'NONE',  ( -99.37424697185159062, -281.0970458832503027, -228.7505034914514965 ) ) ;
#55701=CARTESIAN_POINT ( 'NONE',  ( 24.43040069887143417, -287.1531027544596100, -309.7008689654628597 ) ) ;
#55703=CARTESIAN_POINT ( 'NONE',  ( -50.19781756788521676, -289.8878837452321022, -196.4711938357012286 ) ) ;
#55704=CARTESIAN_POINT ( 'NONE',  ( -107.5886556134111913, -275.3214365662247474, -283.9876634089608274 ) ) ;
#55705=CARTESIAN_POINT ( 'NONE',  ( 15.07801039995889347, -286.3246022718897734, -219.4674799734574151 ) ) ;
#55707=CARTESIAN_POINT ( 'NONE',  ( 32.18438806766314286, -282.9127591946071334, -303.0278025205892618 ) ) ;
#55708=CARTESIAN_POINT ( 'NONE',  ( -108.1454784106161782, -289.9893077222147326, -240.7023049033719531 ) ) ;
#55709=CARTESIAN_POINT ( 'NONE',  ( -39.58434629786869152, -281.6245873055125344, -194.1812092771705238 ) ) ;
#55710=CARTESIAN_POINT ( 'NONE',  ( -113.7386667343605069, -279.8157304895464677, -274.4601135827386997 ) ) ;
#55711=CARTESIAN_POINT ( 'NONE',  ( 15.82440590370200795, -282.1063148144999104, -320.4576903719632242 ) ) ;
#55712=CARTESIAN_POINT ( 'NONE',  ( 36.07400187443877826, -277.3546180322813939, -254.9643979733300796 ) ) ;
#55713=CARTESIAN_POINT ( 'NONE',  ( 4.227299072872228614, -294.5087312939130015, -335.2391569669870250 ) ) ;
#55714=CARTESIAN_POINT ( 'NONE',  ( -105.0376438474083614, -288.9874518093317306, -238.9110622825188273 ) ) ;
#55715=CARTESIAN_POINT ( 'NONE',  ( -69.38026857188837937, -296.5406205986563464, -204.4236005376833134 ) ) ;
#55718=CARTESIAN_POINT ( 'NONE',  ( -111.7572433318797920, -286.4287678944498907, -273.7271644540815601 ) ) ;
#55719=CARTESIAN_POINT ( 'NONE',  ( -39.21796628501986959, -293.1088215601851061, -193.6802010814483026 ) ) ;
#55720=CARTESIAN_POINT ( 'NONE',  ( 22.67319087874643557, -282.7844968492826183, -312.0996556395778612 ) ) ;
#55721=CARTESIAN_POINT ( 'NONE',  ( 37.06014482014440148, -274.3736905368810426, -251.4617613254791024 ) ) ;
#55722=CARTESIAN_POINT ( 'NONE',  ( -73.39327764319359915, -292.2381881952337608, -202.4227762886041830 ) ) ;
#55723=CARTESIAN_POINT ( 'NONE',  ( -110.5218504365429482, -282.9436818642863614, -250.5434911029181251 ) ) ;
#55724=CARTESIAN_POINT ( 'NONE',  ( -37.79916431218168071, -292.3798483090299101, -193.3836211527325872 ) ) ;
#55725=CARTESIAN_POINT ( 'NONE',  ( 27.67503360213356345, -287.4326100166892957, -237.0094317225492944 ) ) ;
#55728=CARTESIAN_POINT ( 'NONE',  ( 65.08017568742300796, 46.23336141765577878, -315.3328154015194400 ) ) ;
#55729=CARTESIAN_POINT ( 'NONE',  ( -27.44268967638380730, -284.4488165136957036, -346.0758614227595444 ) ) ;
#55730=CARTESIAN_POINT ( 'NONE',  ( -85.28047601435909542, -288.9094976428777386, -210.1954327657594206 ) ) ;
#55732=CARTESIAN_POINT ( 'NONE',  ( 34.53102223102401780, -280.6630023714232607, -284.8650735297037500 ) ) ;
#55733=CARTESIAN_POINT ( 'NONE',  ( 22.62185884198586550, -275.8662042734623014, -318.6532404526579398 ) ) ;
#55734=CARTESIAN_POINT ( 'NONE',  ( -21.83886583921823643, -282.2513104852705510, -197.0980541976623215 ) ) ;
#55735=CARTESIAN_POINT ( 'NONE',  ( 155.3744588886772533, 204.7076335705557995, -215.6431656911598509 ) ) ;
#55736=CARTESIAN_POINT ( 'NONE',  ( 38.82581658908117106, -280.0501020718857603, -264.2688533097283994 ) ) ;
#55737=CARTESIAN_POINT ( 'NONE',  ( -110.0326981478991826, -282.3527207339477627, -287.3836503301616858 ) ) ;
#55738=CARTESIAN_POINT ( 'NONE',  ( -113.1122788582135001, -298.3931845793690627, -263.9781883939792806 ) ) ;
#55739=CARTESIAN_POINT ( 'NONE',  ( 34.27556952650019895, -293.8539723999066382, -255.9058376649994102 ) ) ;
#55741=CARTESIAN_POINT ( 'NONE',  ( -55.11551891749013521, -290.5035561635493195, -199.0495842573903928 ) ) ;
#55742=CARTESIAN_POINT ( 'NONE',  ( -28.60436878489555568, -277.5956510857978401, -346.8147002688712064 ) ) ;
#55743=CARTESIAN_POINT ( 'NONE',  ( -99.28047840515753819, -273.0853839058438552, -231.7270948223558094 ) ) ;
#55745=CARTESIAN_POINT ( 'NONE',  ( -3.948224698501486163, -273.4026288294535902, -201.3077763909095950 ) ) ;
#55749=CARTESIAN_POINT ( 'NONE',  ( -8.359437159206827062, -283.7432030591600096, -337.6979912946849822 ) ) ;
#55750=CARTESIAN_POINT ( 'NONE',  ( 37.78931172455114051, -283.1638641883933474, -258.6492710758498106 ) ) ;
#55751=CARTESIAN_POINT ( 'NONE',  ( -110.6259620222402731, -283.6038201957822480, -270.8991039316575211 ) ) ;
#55752=CARTESIAN_POINT ( 'NONE',  ( 32.82876002637679846, -273.6500458308333350, -247.3372971107000922 ) ) ;
#55753=CARTESIAN_POINT ( 'NONE',  ( 3.361782054203298120, -282.4656345588975910, -208.2181152117511544 ) ) ;
#55754=CARTESIAN_POINT ( 'NONE',  ( -7.242007727162001807, -275.1298703312037901, -337.6271292472314940 ) ) ;
#55756=CARTESIAN_POINT ( 'NONE',  ( 3.089007127703217392, -275.6885724997914622, -209.1483183521881131 ) ) ;
#55758=CARTESIAN_POINT ( 'NONE',  ( -95.08268006545570472, -278.6674674094970214, -321.0576470220410670 ) ) ;
#55762=CARTESIAN_POINT ( 'NONE',  ( -111.0124335009993786, -286.1870216109697367, -288.1057534714771009 ) ) ;
#55763=CARTESIAN_POINT ( 'NONE',  ( -5.480408186216903843, -293.8191100215200890, -336.2343521740498886 ) ) ;
#55764=CARTESIAN_POINT ( 'NONE',  ( -37.50970520695263843, -288.4027580212027715, -347.2720563524545128 ) ) ;
#55765=CARTESIAN_POINT ( 'NONE',  ( -86.38102030887576177, -283.6005606901758824, -214.8569168338974293 ) ) ;
#55766=CARTESIAN_POINT ( 'NONE',  ( -107.9624628954410781, -282.8548056065602623, -291.0963094781445193 ) ) ;
#55767=CARTESIAN_POINT ( 'NONE',  ( -15.57473655852678718, -287.0065720128536668, -341.1548522733850746 ) ) ;
#55769=CARTESIAN_POINT ( 'NONE',  ( -110.0074938962367526, -285.8928315151327411, -260.0260843109732605 ) ) ;
#55770=CARTESIAN_POINT ( 'NONE',  ( 37.62310905036242303, -273.5983726887791931, -273.9737064408737979 ) ) ;
#55771=CARTESIAN_POINT ( 'NONE',  ( -7.635997141478554795, -284.8348229458724745, -200.1337411741459107 ) ) ;
#55772=CARTESIAN_POINT ( 'NONE',  ( -111.1748427600444558, -298.7215197931117245, -257.1828138500309251 ) ) ;
#55773=CARTESIAN_POINT ( 'NONE',  ( -33.78790323397614515, -284.0966204425338901, -195.2785037753886854 ) ) ;
#55774=CARTESIAN_POINT ( 'NONE',  ( 19.85228082211398259, -281.8492405191142325, -224.6199221954164216 ) ) ;
#55775=CARTESIAN_POINT ( 'NONE',  ( -29.15101971653988500, -290.9488840420743259, -345.1324524934789792 ) ) ;
#55777=FACE_OUTER_BOUND ( 'NONE', #84697, .T. ) ;
#55778=CARTESIAN_POINT ( 'NONE',  ( -58.42561724735296025, -297.2426359752225835, -342.9744673645919875 ) ) ;
#55779=CARTESIAN_POINT ( 'NONE',  ( -82.47157427380329864, -277.4361608080855603, -210.3935417485051858 ) ) ;
#55780=CARTESIAN_POINT ( 'NONE',  ( 33.18025448408185696, -292.3597320987174726, -239.8518941690257407 ) ) ;
#55781=CARTESIAN_POINT ( 'NONE',  ( -94.57576155651388206, -294.2995129234390674, -316.9717853151980762 ) ) ;
#55782=CARTESIAN_POINT ( 'NONE',  ( -87.85751897368534458, -278.0132771434929850, -216.9110740695190032 ) ) ;
#55783=CARTESIAN_POINT ( 'NONE',  ( -100.4893558085904743, -271.1655393221718100, -230.9442715989578971 ) ) ;
#55784=CARTESIAN_POINT ( 'NONE',  ( 33.09694854689596610, -294.5896179906439443, -249.2182908589441297 ) ) ;
#55785=CARTESIAN_POINT ( 'NONE',  ( -110.4683760289727132, -293.2662352645559167, -253.7030783399848985 ) ) ;
#55786=CARTESIAN_POINT ( 'NONE',  ( -101.7209603822269912, -295.5738542108901470, -229.3974926409373438 ) ) ;
#55787=CARTESIAN_POINT ( 'NONE',  ( 35.73587712130937177, -291.5269599033745180, -249.4895906788872253 ) ) ;
#55788=CARTESIAN_POINT ( 'NONE',  ( -109.7555292035626309, -291.8060000616287084, -283.4612048821228427 ) ) ;
#55791=CARTESIAN_POINT ( 'NONE',  ( -110.4983976614188919, -291.3439824565651861, -271.1973789680909022 ) ) ;
#55793=CARTESIAN_POINT ( 'NONE',  ( -111.1552297526095003, -291.4992625893619334, -290.8445640704211996 ) ) ;
#55794=CARTESIAN_POINT ( 'NONE',  ( -1.886548434290350240, -278.5395588520241290, -203.8679677830192531 ) ) ;
#55795=CARTESIAN_POINT ( 'NONE',  ( 27.48653718474616525, -293.0957602275715885, -236.8007299199687168 ) ) ;
#55796=CARTESIAN_POINT ( 'NONE',  ( -28.22500312982331039, -280.1646684249916461, -193.8491002969554984 ) ) ;
#55797=CARTESIAN_POINT ( 'NONE',  ( -114.1875369891244247, -284.1519321946227024, -275.7120810180312560 ) ) ;
#55798=CARTESIAN_POINT ( 'NONE',  ( 27.26633376575570367, -286.0588070545921369, -308.2236728744064180 ) ) ;
#55799=CARTESIAN_POINT ( 'NONE',  ( -93.50896925536522986, -282.0114961195919250, -318.9201793785103405 ) ) ;
#55800=CARTESIAN_POINT ( 'NONE',  ( -3.943430770372944760, -278.9645314803108249, -201.7372293118942821 ) ) ;
#55801=CARTESIAN_POINT ( 'NONE',  ( -46.45507292069262206, -284.8593993161610456, -194.2136364376552820 ) ) ;
#55803=CARTESIAN_POINT ( 'NONE',  ( 36.22349847479316765, -295.2290441538630716, -276.2434617587404091 ) ) ;
#55804=CARTESIAN_POINT ( 'NONE',  ( 17.65280880277210329, -276.2447126287162860, -217.2360527939434292 ) ) ;
#55805=CARTESIAN_POINT ( 'NONE',  ( -48.61529096533158167, -276.8662340104509667, -342.5581641288240462 ) ) ;
#55806=CARTESIAN_POINT ( 'NONE',  ( -111.5414034733405231, -290.4610346717873313, -290.9379016961150342 ) ) ;
#55807=CARTESIAN_POINT ( 'NONE',  ( -3.559017702572665254, -280.6897044565262718, -337.9628060080183900 ) ) ;
#55808=CARTESIAN_POINT ( 'NONE',  ( 9.006989620723835799, -291.7648262048850825, -213.5925334579890773 ) ) ;
#55809=CARTESIAN_POINT ( 'NONE',  ( -110.0365941876441696, -294.3143545456031234, -288.8644052524561516 ) ) ;
#55812=CARTESIAN_POINT ( 'NONE',  ( -36.19888313780195688, -291.5744784292485292, -197.2960307922057268 ) ) ;
#55814=CARTESIAN_POINT ( 'NONE',  ( 7.399455738971487229, -291.9094976428775681, -326.5171145203363494 ) ) ;
#55815=CARTESIAN_POINT ( 'NONE',  ( -81.74539468072137538, -294.6989818203433060, -333.0449921331582459 ) ) ;
#55816=CARTESIAN_POINT ( 'NONE',  ( 16.36453107020616926, -278.9441997284798731, -216.8464740409250453 ) ) ;
#55817=CARTESIAN_POINT ( 'NONE',  ( -21.10505758099044371, -287.5714525714565184, -195.5970242595604986 ) ) ;
#55818=CARTESIAN_POINT ( 'NONE',  ( 34.52131555760914239, -287.5547708797462292, -283.1949397468496841 ) ) ;
#55819=CARTESIAN_POINT ( 'NONE',  ( -54.09289418273807115, -278.7911472558761830, -342.1779847956091771 ) ) ;
#55820=CARTESIAN_POINT ( 'NONE',  ( -94.35464198576957529, -293.9024660101249538, -318.5615386243209741 ) ) ;
#55821=CARTESIAN_POINT ( 'NONE',  ( -73.78206468869193202, -297.3032420467771431, -334.7821847612454462 ) ) ;
#55822=CARTESIAN_POINT ( 'NONE',  ( -64.49423303950477759, -276.2094338642514799, -338.6050565531623420 ) ) ;
#55825=CARTESIAN_POINT ( 'NONE',  ( -112.2861918467459645, -295.9982331894827894, -287.9984599004405368 ) ) ;
#55826=CARTESIAN_POINT ( 'NONE',  ( -110.7000149349150462, -292.6396919553939142, -257.4222166310048578 ) ) ;
#55827=CARTESIAN_POINT ( 'NONE',  ( 200.9738101188480641, 294.0933875133407582, -53.99999999999736389 ) ) ;
#55828=CARTESIAN_POINT ( 'NONE',  ( 19.59809741626572688, -288.8508133312125779, -316.2059881883614025 ) ) ;
#55831=CARTESIAN_POINT ( 'NONE',  ( -38.15535180422752148, -279.1009419465214592, -193.6007233445317581 ) ) ;
#55832=CARTESIAN_POINT ( 'NONE',  ( -96.42776434157040910, -296.5404914507276430, -319.5969309025309713 ) ) ;
#55833=CARTESIAN_POINT ( 'NONE',  ( -107.2186457609142565, -289.0702917503227809, -241.0777106136807788 ) ) ;
#55835=CARTESIAN_POINT ( 'NONE',  ( -36.90127381467026169, -298.3908043557193537, -193.3822376128566702 ) ) ;
#55836=CARTESIAN_POINT ( 'NONE',  ( 34.85953520503804981, -294.0336780712257223, -281.6020136788554282 ) ) ;
#55840=CARTESIAN_POINT ( 'NONE',  ( -17.88229110778965136, -290.3257672423472400, -344.1448502786595327 ) ) ;
#55841=CARTESIAN_POINT ( 'NONE',  ( -115.3430155898818299, -281.2662352645559167, -252.5904736702033517 ) ) ;
#55844=CARTESIAN_POINT ( 'NONE',  ( 25.84183455916705086, -281.4808017252806280, -314.2152407590183429 ) ) ;
#55845=CARTESIAN_POINT ( 'NONE',  ( -84.83047191448920898, -287.3962458681714907, -212.4591364090152013 ) ) ;
#55847=CARTESIAN_POINT ( 'NONE',  ( 38.50338223247301528, -286.2491977846910913, -280.0664877549826883 ) ) ;
#55848=CARTESIAN_POINT ( 'NONE',  ( -79.87671474844671593, -271.4756853532445007, -208.7287062667988948 ) ) ;
#55849=CARTESIAN_POINT ( 'NONE',  ( -36.74868521505418073, -275.9798131421405856, -195.9108166195481147 ) ) ;
#55850=CARTESIAN_POINT ( 'NONE',  ( -99.32295929599442275, -288.0705370889169217, -311.6109972932421783 ) ) ;
#55851=CARTESIAN_POINT ( 'NONE',  ( -69.75079384670668503, -279.3346533238908478, -338.8585765529960554 ) ) ;
#55853=CARTESIAN_POINT ( 'NONE',  ( -79.05486759071510505, -279.4718180145512747, -210.4527574622263728 ) ) ;
#55854=CARTESIAN_POINT ( 'NONE',  ( -30.24424277496249047, -279.4927526733891341, -197.5541204920621681 ) ) ;
#55855=CARTESIAN_POINT ( 'NONE',  ( 38.61611732443666511, -276.4989896970977270, -259.7827212467331606 ) ) ;
#55856=CARTESIAN_POINT ( 'NONE',  ( -53.66084412209648491, -278.6423028466743972, -195.4623654345158741 ) ) ;
#55857=CARTESIAN_POINT ( 'NONE',  ( -14.16128100611320306, -91.36119643908550358, -357.2170007693700882 ) ) ;
#55858=CARTESIAN_POINT ( 'NONE',  ( -93.97978581159480882, -274.2004802261873238, -218.5252275717888040 ) ) ;
#55859=CARTESIAN_POINT ( 'NONE',  ( -57.25379985901823687, -299.2255164674996877, -196.5355697911905963 ) ) ;
#55860=CARTESIAN_POINT ( 'NONE',  ( 10.59707575819634329, -283.1948066931273047, -210.1954327657594490 ) ) ;
#55861=EDGE_LOOP ( 'NONE', ( #24285, #50689, #49205, #59227 ) ) ;
#55863=CARTESIAN_POINT ( 'NONE',  ( 19.76288963607669302, -289.2790021743219313, -316.3316727168393641 ) ) ;
#55864=CARTESIAN_POINT ( 'NONE',  ( 29.23279321469740921, -288.8302933671461687, -233.6212629989304901 ) ) ;
#55865=CARTESIAN_POINT ( 'NONE',  ( -90.67279597412355940, -289.1816131803250869, -320.4319183225489951 ) ) ;
#55866=CARTESIAN_POINT ( 'NONE',  ( -105.7323232406256324, -283.6038696310185969, -305.7229403694566940 ) ) ;
#55867=CARTESIAN_POINT ( 'NONE',  ( -51.96617292990010384, -278.2618729916962366, -197.9723508188855590 ) ) ;
#55868=CARTESIAN_POINT ( 'NONE',  ( 18.69325183354095898, -288.7299117239803650, -221.6687197992358165 ) ) ;
#55869=CARTESIAN_POINT ( 'NONE',  ( 36.25740623410334962, -280.0807058659170252, -274.0866103614196732 ) ) ;
#55870=CARTESIAN_POINT ( 'NONE',  ( -66.27919769689943053, -280.9803944930607713, -202.7910034938128376 ) ) ;
#55871=CARTESIAN_POINT ( 'NONE',  ( -41.85412637857432117, -277.6028586809467242, -343.2957823925473804 ) ) ;
#55872=CARTESIAN_POINT ( 'NONE',  ( -97.85542198797053004, -288.7165946713528797, -317.3302374858305939 ) ) ;
#55873=CARTESIAN_POINT ( 'NONE',  ( -30.21966086357525683, -283.7670395628373967, -346.8688651529612912 ) ) ;
#55874=CARTESIAN_POINT ( 'NONE',  ( -111.4305179371361731, -284.7843327317326612, -291.1065748104892350 ) ) ;
#55875=CARTESIAN_POINT ( 'NONE',  ( -26.74067808226551080, -283.0803734113878249, -342.6385788490022151 ) ) ;
#55878=CARTESIAN_POINT ( 'NONE',  ( -108.3250529612868007, -292.7547362850664285, -243.7224436749581855 ) ) ;
#55879=CARTESIAN_POINT ( 'NONE',  ( -42.00705088205833704, -290.6793331058134982, -193.9966447276455312 ) ) ;
#55880=CARTESIAN_POINT ( 'NONE',  ( 20.87584843434727944, -273.9878481103862669, -225.9093399019967023 ) ) ;
#55881=CARTESIAN_POINT ( 'NONE',  ( 17.48304448391924737, -293.6427124877519077, -324.3586428718817842 ) ) ;
#55882=CARTESIAN_POINT ( 'NONE',  ( -95.50966863292985920, -288.4003599626506116, -315.6274541830374005 ) ) ;
#55883=CARTESIAN_POINT ( 'NONE',  ( 31.52024291141157519, -292.1514989223406360, -297.6306795168488293 ) ) ;
#55884=CARTESIAN_POINT ( 'NONE',  ( -110.0139457998354118, -291.6210493910559762, -280.7407214309300798 ) ) ;
#55886=CARTESIAN_POINT ( 'NONE',  ( -97.41158021147037971, -291.9386487216985984, -315.2890294410007073 ) ) ;
#55887=CARTESIAN_POINT ( 'NONE',  ( 5.473371315473700705, -290.6302035960407011, -208.5800684491783841 ) ) ;
#55888=CARTESIAN_POINT ( 'NONE',  ( -14.97970168342837205, -296.7627957996746204, -342.0032791716342899 ) ) ;
#55889=CARTESIAN_POINT ( 'NONE',  ( 17.05738341949641068, -287.7933754856827591, -221.3102863981775954 ) ) ;
#55890=CARTESIAN_POINT ( 'NONE',  ( -63.60126968552361149, -297.3938025512567265, -340.7916755050466122 ) ) ;
#55891=CARTESIAN_POINT ( 'NONE',  ( 36.33185452959686756, -277.3289541461293197, -254.4694129795140327 ) ) ;
#55892=CARTESIAN_POINT ( 'NONE',  ( -62.78192564562182554, -296.9263962180383487, -197.8562647251423527 ) ) ;
#55893=CARTESIAN_POINT ( 'NONE',  ( -56.88908866994516700, -275.5474131657332464, -341.7997376742808342 ) ) ;
#55894=CARTESIAN_POINT ( 'NONE',  ( -36.97720910188893839, -278.1365987337397883, -195.9220062992334590 ) ) ;
#55895=CARTESIAN_POINT ( 'NONE',  ( -36.74819187013572730, -275.2648506555660788, -196.9539611793013307 ) ) ;
#55896=CARTESIAN_POINT ( 'NONE',  ( -39.68980033698543508, -296.5074572549635263, -343.9254086251661420 ) ) ;
#55898=CARTESIAN_POINT ( 'NONE',  ( -109.2062116672338732, -297.5363869913909411, -256.5796213035073379 ) ) ;
#55900=CARTESIAN_POINT ( 'NONE',  ( 144.2857639756989272, -299.5541904835127980, -195.3611179825600175 ) ) ;
#55901=CARTESIAN_POINT ( 'NONE',  ( 37.34841062809199030, -285.4445980340938149, -260.3714153990554792 ) ) ;
#55902=CARTESIAN_POINT ( 'NONE',  ( -96.28011415179295795, -272.9896300714245854, -227.2043692953074014 ) ) ;
#55903=CARTESIAN_POINT ( 'NONE',  ( 34.85422980127450643, -287.2136738447925381, -243.5889738466200924 ) ) ;
#55905=CARTESIAN_POINT ( 'NONE',  ( -43.18492493439285340, -288.7907554321525367, -347.1178832569394217 ) ) ;
#55906=CARTESIAN_POINT ( 'NONE',  ( -70.03866069211196077, -299.6034460271838498, -202.4691775345005453 ) ) ;
#55907=CARTESIAN_POINT ( 'NONE',  ( -7.274496013806282413, -292.6567565528593491, -338.9023397666148867 ) ) ;
#55908=CARTESIAN_POINT ( 'NONE',  ( 34.43302058299196489, -281.0973585484160822, -297.7937315470803128 ) ) ;
#55909=CARTESIAN_POINT ( 'NONE',  ( -54.49178911615187815, -286.7666405000204577, -345.3538533559490702 ) ) ;
#55910=CARTESIAN_POINT ( 'NONE',  ( -87.92197074771574705, -277.3452524989666585, -214.9147161604864493 ) ) ;
#55911=CARTESIAN_POINT ( 'NONE',  ( -90.89292050906632880, -288.6280399794289337, -320.6289542331822986 ) ) ;
#55913=CARTESIAN_POINT ( 'NONE',  ( -105.8856430268801887, -288.1516246467788847, -300.9316883930976587 ) ) ;
#55914=CARTESIAN_POINT ( 'NONE',  ( -95.16870256805567863, -274.7108019603028310, -224.6802079267853856 ) ) ;
#55915=CARTESIAN_POINT ( 'NONE',  ( 32.62606933562828715, -282.5827397648077977, -239.6508993634868148 ) ) ;
#55916=CARTESIAN_POINT ( 'NONE',  ( -72.49048407444017528, -295.6097756893146880, -203.6479357346821644 ) ) ;
#55917=CARTESIAN_POINT ( 'NONE',  ( 21.00990313595386993, -282.1683262619324637, -314.2462292977136826 ) ) ;
#55918=CARTESIAN_POINT ( 'NONE',  ( -108.3742201476035518, -296.3392501628699165, -300.2208348617602383 ) ) ;
#55919=CARTESIAN_POINT ( 'NONE',  ( -92.47153030126679596, -274.6682450133892530, -221.6161003592695522 ) ) ;
#55920=CARTESIAN_POINT ( 'NONE',  ( 38.14058268163777399, -285.5754942089768065, -265.9277254572482434 ) ) ;
#55921=CARTESIAN_POINT ( 'NONE',  ( -17.54506600210016032, -282.3077298343403641, -198.0209913362684517 ) ) ;
#55922=CARTESIAN_POINT ( 'NONE',  ( -108.2354701892585922, -271.7201905374424769, -251.5038136496105494 ) ) ;
#55925=CARTESIAN_POINT ( 'NONE',  ( -111.2441444686217409, -286.6675229615570970, -259.8599026558893001 ) ) ;
#55927=CARTESIAN_POINT ( 'NONE',  ( 36.57525178469694538, -279.4809262143061233, -305.9938812882205070 ) ) ;
#55928=CARTESIAN_POINT ( 'NONE',  ( 30.39587602696987290, -275.2204084354752354, -306.7471127574326033 ) ) ;
#55929=CARTESIAN_POINT ( 'NONE',  ( -85.29845084291568469, -285.2492099288584200, -326.3151867489012261 ) ) ;
#55930=CARTESIAN_POINT ( 'NONE',  ( -92.98987905329120451, -285.2569901151141494, -322.7433206337930187 ) ) ;
#55931=CARTESIAN_POINT ( 'NONE',  ( -40.26545599562581401, -281.8846417625223353, -343.6999355166549321 ) ) ;
#55932=CARTESIAN_POINT ( 'NONE',  ( 12.61967677588809167, -282.7489176715701547, -214.4248912238800813 ) ) ;
#55933=CARTESIAN_POINT ( 'NONE',  ( -66.22918976118340595, -273.8509994291147791, -198.9710907124845392 ) ) ;
#55934=CARTESIAN_POINT ( 'NONE',  ( 25.32813594469280005, -274.7926116731607635, -225.6005275951170574 ) ) ;
#55935=CARTESIAN_POINT ( 'NONE',  ( -106.2865849365744708, -298.1035589174763913, -298.4309782289709005 ) ) ;
#55938=CARTESIAN_POINT ( 'NONE',  ( -100.5066118230988934, -295.2513606600918479, -228.4985345894234570 ) ) ;
#55939=CARTESIAN_POINT ( 'NONE',  ( 18.35125672540491948, -275.7316529746526612, -317.6504719508592416 ) ) ;
#55940=CARTESIAN_POINT ( 'NONE',  ( -52.31554381620688332, -287.6179290135529527, -197.8783061155932330 ) ) ;
#55941=CARTESIAN_POINT ( 'NONE',  ( 35.71161274853539425, -295.3535080424982766, -292.5838881597506997 ) ) ;
#55942=CARTESIAN_POINT ( 'NONE',  ( 23.72179193499144745, -295.3765905230803241, -316.6132385493590391 ) ) ;
#55944=CARTESIAN_POINT ( 'NONE',  ( -108.3180105222826342, -292.8595474917478327, -246.6463169331190102 ) ) ;
#55945=CARTESIAN_POINT ( 'NONE',  ( -72.98095372644304746, -277.5785202583151090, -204.5593548495735661 ) ) ;
#55946=CARTESIAN_POINT ( 'NONE',  ( -102.0758771461041476, -280.9659075920111491, -233.6078797385226551 ) ) ;
#55947=CARTESIAN_POINT ( 'NONE',  ( -87.47752126717529109, -293.8381145249664428, -325.3857818550354182 ) ) ;
#55948=CARTESIAN_POINT ( 'NONE',  ( 10.72751330863799701, -284.2566703096534297, -328.9922918666186433 ) ) ;
#55949=CARTESIAN_POINT ( 'NONE',  ( -65.19799313359399662, -284.5998147868286878, -202.4966679312256019 ) ) ;
#55950=CARTESIAN_POINT ( 'NONE',  ( -107.7075741586806004, -267.3548955105460436, -306.6422084984729395 ) ) ;
#55952=CARTESIAN_POINT ( 'NONE',  ( -107.7826725225565525, -283.9641996549107716, -289.6477982820007924 ) ) ;
#55954=CARTESIAN_POINT ( 'NONE',  ( 37.02812134833334312, -282.3965876746442518, -251.6362103877525840 ) ) ;
#55955=CARTESIAN_POINT ( 'NONE',  ( -110.2101890171688723, -272.9572434417630120, -264.9161015990332544 ) ) ;
#55956=CARTESIAN_POINT ( 'NONE',  ( -87.47840982099886276, -284.1659497068868063, -212.3744229478787133 ) ) ;
#55957=CARTESIAN_POINT ( 'NONE',  ( -90.90261130641086140, -280.2559220546347092, -215.2956475704461070 ) ) ;
#55958=CARTESIAN_POINT ( 'NONE',  ( -39.91996080952217341, -278.6040766945079667, -346.6371661126491972 ) ) ;
#55959=CARTESIAN_POINT ( 'NONE',  ( -62.02277691988539488, -280.3910522545137951, -197.4753124099462696 ) ) ;
#55960=CARTESIAN_POINT ( 'NONE',  ( 7.450504543161054372, -272.1952119285918457, -214.2458315076590907 ) ) ;
#55961=CARTESIAN_POINT ( 'NONE',  ( -106.8288633700993842, -263.1380580373908060, -317.6964085897507744 ) ) ;
#55963=CARTESIAN_POINT ( 'NONE',  ( 21.27606504587327407, -276.9115181615392771, -223.8219603609496460 ) ) ;
#55964=CARTESIAN_POINT ( 'NONE',  ( -40.17672028908389592, -139.3485780022602114, -364.5271839380368988 ) ) ;
#55966=CARTESIAN_POINT ( 'NONE',  ( -110.4942328733011010, -276.7646804713084521, -255.4459848794400898 ) ) ;
#55967=CARTESIAN_POINT ( 'NONE',  ( 8.225115480596734585, -294.4256391158502311, -209.4872439545429756 ) ) ;
#55968=CARTESIAN_POINT ( 'NONE',  ( -88.57920399699580116, -295.1424681792105389, -322.5725643634546600 ) ) ;
#55969=CARTESIAN_POINT ( 'NONE',  ( -113.3002979947120679, -289.9066060351497072, -282.6011471253438572 ) ) ;
#55971=CARTESIAN_POINT ( 'NONE',  ( -112.0207258588586399, -295.3314643056204432, -254.1245355009379523 ) ) ;
#55972=CARTESIAN_POINT ( 'NONE',  ( -9.169343535973261794, -284.8266026337799417, -202.1363265868821202 ) ) ;
#55973=CARTESIAN_POINT ( 'NONE',  ( -100.7792367118623105, -292.9347134587859500, -231.8053864879299510 ) ) ;
#55974=CARTESIAN_POINT ( 'NONE',  ( -110.7217342482675235, -285.9316996899287915, -265.4488170674724756 ) ) ;
#55976=CARTESIAN_POINT ( 'NONE',  ( -69.53545040790464782, -292.5799643079080283, -200.6590684102577882 ) ) ;
#55977=CARTESIAN_POINT ( 'NONE',  ( -65.33347925078153651, -283.9205091120809357, -337.8613834636599904 ) ) ;
#55978=CARTESIAN_POINT ( 'NONE',  ( -94.36630442429415666, -294.6493489821700109, -321.5294999101631106 ) ) ;
#55979=CARTESIAN_POINT ( 'NONE',  ( -113.1990069752303185, -291.2015767068866694, -282.6015353977554128 ) ) ;
#55980=CARTESIAN_POINT ( 'NONE',  ( -113.2983005987443050, -290.8911414489775780, -282.6135360386335833 ) ) ;
#55981=CARTESIAN_POINT ( 'NONE',  ( 24.23948716713388762, -288.2608561698000358, -309.5626150944148094 ) ) ;
#55984=CARTESIAN_POINT ( 'NONE',  ( -93.71639224285308956, -297.7143456237691339, -320.9986143411068724 ) ) ;
#55985=CARTESIAN_POINT ( 'NONE',  ( -43.23495037039796074, -296.6641745611853480, -194.0287110980780767 ) ) ;
#55986=CARTESIAN_POINT ( 'NONE',  ( -72.23128332299555154, -278.6372576719850827, -205.9707038432285344 ) ) ;
#55987=CARTESIAN_POINT ( 'NONE',  ( 29.89680538609862026, -274.5734307707119228, -232.8548872660012421 ) ) ;
#55988=CARTESIAN_POINT ( 'NONE',  ( -110.9350641024688997, -294.9818793123391742, -274.1983734775977268 ) ) ;
#55989=CARTESIAN_POINT ( 'NONE',  ( 10.47749449157027790, -278.2439866612750734, -327.1430702514073801 ) ) ;
#55990=CARTESIAN_POINT ( 'NONE',  ( 21.67773767129911633, -273.0688328519118500, -225.3116234614367386 ) ) ;
#55991=CARTESIAN_POINT ( 'NONE',  ( -68.67297359981033367, -296.6784032147823496, -336.7487265291185281 ) ) ;
#55992=CARTESIAN_POINT ( 'NONE',  ( -72.25975483507748720, -296.6052505806879367, -334.8343906807415920 ) ) ;
#55994=CARTESIAN_POINT ( 'NONE',  ( -95.88358803708518963, -297.4890531626940060, -319.1593432995440480 ) ) ;
#55995=CARTESIAN_POINT ( 'NONE',  ( -111.4460249503558344, -270.7505508581946287, -256.4098452757740461 ) ) ;
#55996=CARTESIAN_POINT ( 'NONE',  ( -49.71412802039538548, -292.5417297973257860, -198.2624042794496404 ) ) ;
#55997=CARTESIAN_POINT ( 'NONE',  ( -78.76312769857507590, -274.3119664689808133, -205.6430821792482391 ) ) ;
#55998=CARTESIAN_POINT ( 'NONE',  ( -110.0037841511857977, -288.9734550269866986, -282.0850863145746530 ) ) ;
#56000=CARTESIAN_POINT ( 'NONE',  ( -81.22044027451509862, -273.9659596949470597, -207.0970052568395658 ) ) ;
#56001=CARTESIAN_POINT ( 'NONE',  ( -107.6220062574573575, -296.6235284075772256, -290.1794442787860362 ) ) ;
#56002=CARTESIAN_POINT ( 'NONE',  ( -74.22535347838116593, -281.5442461561903542, -204.6496051451285325 ) ) ;
#56003=CARTESIAN_POINT ( 'NONE',  ( 32.72804225596879490, -279.8427345702752973, -239.6441931085220176 ) ) ;
#56004=CARTESIAN_POINT ( 'NONE',  ( -7.931305937635153569, -276.0254187580629264, -341.4270648641387993 ) ) ;
#56005=CARTESIAN_POINT ( 'NONE',  ( 22.26243476972170754, -279.3095750331083877, -222.8662941098490933 ) ) ;
#56006=CARTESIAN_POINT ( 'NONE',  ( 28.15169309927801677, -280.0435018229886737, -307.3540410067049606 ) ) ;
#56007=CARTESIAN_POINT ( 'NONE',  ( -27.19108800622527866, -272.7582728492885735, -197.4240066745856268 ) ) ;
#56008=CARTESIAN_POINT ( 'NONE',  ( -13.27255544842608082, -278.7398390813743276, -341.4481691860847263 ) ) ;
#56011=CARTESIAN_POINT ( 'NONE',  ( -90.90513193883295173, -295.5443093140505084, -216.4636896091547271 ) ) ;
#56012=CARTESIAN_POINT ( 'NONE',  ( -22.19378902478616311, -292.2408841875071630, -194.8114887592158198 ) ) ;
#56013=CARTESIAN_POINT ( 'NONE',  ( 0.1551213403316603068, -278.5547186166668894, -335.5662848355707411 ) ) ;
#56014=CARTESIAN_POINT ( 'NONE',  ( 23.10787926403396852, -272.9466195775318056, -225.9668728316694057 ) ) ;
#56015=DIRECTION ( 'NONE',  ( 0.000000000000000000, 0.000000000000000000, 1.000000000000000000 ) ) ;
#56016=CARTESIAN_POINT ( 'NONE',  ( 12.74489682270729141, -284.2804808577405993, -327.0050446814506131 ) ) ;
#56019=CARTESIAN_POINT ( 'NONE',  ( 37.66962986651619616, -285.5834618133250160, -272.8124283608974565 ) ) ;
#56022=CARTESIAN_POINT ( 'NONE',  ( -45.14814083827369728, -293.9479929199981711, -343.3926203374080046 ) ) ;
#56023=CARTESIAN_POINT ( 'NONE',  ( -4.019223346084575432, -284.6360237272390350, -204.0250190281032019 ) ) ;
#56025=CARTESIAN_POINT ( 'NONE',  ( -5.950385865498482474, -292.6393662856775109, -338.4756248186760672 ) ) ;
#56026=CARTESIAN_POINT ( 'NONE',  ( -65.60242375132042980, -284.1691266791250996, -199.4666351295204265 ) ) ;
#56027=CARTESIAN_POINT ( 'NONE',  ( -68.88349678279791988, -281.2304653985445384, -203.6411398544783253 ) ) ;
#56028=CARTESIAN_POINT ( 'NONE',  ( -2.417699391155528676, -287.7088322681562431, -202.1678324573639145 ) ) ;
#56029=CARTESIAN_POINT ( 'NONE',  ( 38.51599593232745633, -279.8585754077139995, -275.6134851717976630 ) ) ;
#56030=CARTESIAN_POINT ( 'NONE',  ( 35.65517884072506405, -287.5610568891780758, -271.0361445105027656 ) ) ;
#56032=CARTESIAN_POINT ( 'NONE',  ( -24.79362128576465452, -281.6406575474871374, -197.8495972905729730 ) ) ;
#56033=CARTESIAN_POINT ( 'NONE',  ( 18.08017707397654306, -281.6760748464290032, -222.5818940085184749 ) ) ;
#56034=CARTESIAN_POINT ( 'NONE',  ( 0.6697430067040709423, -288.5361353586789050, -205.2804738438148604 ) ) ;
#56037=CARTESIAN_POINT ( 'NONE',  ( -36.89473150819597436, -297.8909244976909463, -193.3611301614376430 ) ) ;
#56039=CARTESIAN_POINT ( 'NONE',  ( -104.3102276518549019, -292.0951064787559517, -303.3317582684422291 ) ) ;
#56041=CARTESIAN_POINT ( 'NONE',  ( -85.33152481854864391, -275.9090924074130839, -210.2361428286349110 ) ) ;
#56043=CARTESIAN_POINT ( 'NONE',  ( 30.89960074401644263, -273.1375551215259065, -238.7227445224759208 ) ) ;
#56045=CARTESIAN_POINT ( 'NONE',  ( -102.4428027032239470, -294.4295120102975716, -309.9627196893305268 ) ) ;
#56046=CARTESIAN_POINT ( 'NONE',  ( 8.983965382278052303, -298.1551325937431329, -197.3035830641272526 ) ) ;
#56047=CARTESIAN_POINT ( 'NONE',  ( -66.58653162377873969, -290.9622919390602078, -338.0576942310134427 ) ) ;
#56048=CARTESIAN_POINT ( 'NONE',  ( 34.74228035353977617, -283.0938460413431130, -253.5720210866410014 ) ) ;
#56049=CARTESIAN_POINT ( 'NONE',  ( -15.10623445322716663, -290.1951008165304984, -343.5204162540024413 ) ) ;
#56050=CARTESIAN_POINT ( 'NONE',  ( -87.05122025990725376, -291.0424129964769122, -328.5879059861280780 ) ) ;
#56051=CARTESIAN_POINT ( 'NONE',  ( -65.87713355294340545, -287.6791493860777678, -200.9464024555221044 ) ) ;
#56052=CARTESIAN_POINT ( 'NONE',  ( -38.17203572532561395, -280.2086946658774878, -193.3655950781079866 ) ) ;
#56053=CARTESIAN_POINT ( 'NONE',  ( 36.65532809355934063, -291.8268569546354456, -285.6501341635693052 ) ) ;
#56054=CARTESIAN_POINT ( 'NONE',  ( 32.02238942766086183, -280.9552158191860372, -236.8075744291823241 ) ) ;
#56055=CARTESIAN_POINT ( 'NONE',  ( 33.22876386161097173, -277.1100321137354285, -247.1595325974809612 ) ) ;
#56057=CARTESIAN_POINT ( 'NONE',  ( 27.33386217378599881, -283.6233781216987495, -239.1787733560258573 ) ) ;
#56058=CARTESIAN_POINT ( 'NONE',  ( 37.92359159668361457, -273.6596351941662988, -259.9155507374346143 ) ) ;
#56060=CARTESIAN_POINT ( 'NONE',  ( 35.76431847340407444, -281.0724510958451674, -271.3208181675600486 ) ) ;
#56061=CARTESIAN_POINT ( 'NONE',  ( -38.52336472219708696, -278.2717301988474219, -346.9549322820475936 ) ) ;
#56062=CARTESIAN_POINT ( 'NONE',  ( -102.4752169656997580, -274.3287924989739963, -236.2086887407280358 ) ) ;
#56063=CARTESIAN_POINT ( 'NONE',  ( -112.1277792125293615, -283.8281385059705144, -253.0445770638732768 ) ) ;
#56064=CARTESIAN_POINT ( 'NONE',  ( -63.17513472305719091, -293.4711289431203909, -201.0025736617258474 ) ) ;
#56065=CARTESIAN_POINT ( 'NONE',  ( -71.06725443763581040, -275.2145963204682744, -202.0308362257548538 ) ) ;
#56066=CARTESIAN_POINT ( 'NONE',  ( -68.65762688818671222, -274.9642966368102179, -200.5427231659969323 ) ) ;
#56068=CARTESIAN_POINT ( 'NONE',  ( 18.30703445672270036, -276.0572674661329984, -317.6074759759202948 ) ) ;
#56069=CARTESIAN_POINT ( 'NONE',  ( -50.77594290759483187, -297.2243425807369022, -343.9787078956802588 ) ) ;
#56070=CARTESIAN_POINT ( 'NONE',  ( -57.87353748088431615, -283.7863288919468232, -198.3455879892530334 ) ) ;
#56071=CARTESIAN_POINT ( 'NONE',  ( 4.133717683148574018, -292.2610753755764108, -205.4478441155281132 ) ) ;
#56072=CARTESIAN_POINT ( 'NONE',  ( 1.710938404082930742, -274.5476746908430528, -334.0358190628547845 ) ) ;
#56073=CARTESIAN_POINT ( 'NONE',  ( 14.07904642907681314, -289.9450211195631937, -326.6673892184522288 ) ) ;
#56074=CARTESIAN_POINT ( 'NONE',  ( -104.3357715634736422, -289.0719655914077180, -300.2526313965403801 ) ) ;
#56076=CARTESIAN_POINT ( 'NONE',  ( -30.73002346790145722, -290.7087765773584351, -194.1845752282874855 ) ) ;
#56077=CARTESIAN_POINT ( 'NONE',  ( -105.7289510306664653, -290.5619881419297599, -244.6193941095278319 ) ) ;
#56079=CARTESIAN_POINT ( 'NONE',  ( 39.29615340389884182, -288.6824484063742489, -274.3929202436269179 ) ) ;
#56080=CARTESIAN_POINT ( 'NONE',  ( -87.54824253368641962, -279.6614668651365037, -217.2686879053882194 ) ) ;
#56082=CARTESIAN_POINT ( 'NONE',  ( -33.46427230025540211, -293.9247800029913833, -346.9669916583351892 ) ) ;
#56083=CARTESIAN_POINT ( 'NONE',  ( -76.06257783564061015, -286.2008183768584786, -203.8618062814195753 ) ) ;
#56084=CARTESIAN_POINT ( 'NONE',  ( -78.51473750191632917, -285.8471941912260377, -205.3186296776731012 ) ) ;
#56085=CARTESIAN_POINT ( 'NONE',  ( 28.17191445445139664, -282.3236899235331521, -302.7257461959653710 ) ) ;
#56086=CARTESIAN_POINT ( 'NONE',  ( 180.2115114871389210, 254.1752151913870250, -166.7759868809612840 ) ) ;
#56087=CARTESIAN_POINT ( 'NONE',  ( 188.1608565823388801, 271.2200784998753420, -139.0206290322748544 ) ) ;
#56088=CARTESIAN_POINT ( 'NONE',  ( -94.43123972790466780, -238.4150439815195739, -338.5472242393929605 ) ) ;
#56089=CARTESIAN_POINT ( 'NONE',  ( 34.86484249539895330, -274.9084239664247775, -282.4490291555209751 ) ) ;
#56090=CARTESIAN_POINT ( 'NONE',  ( 19.24619231726884649, -273.8147980199998415, -223.7560055679572883 ) ) ;
#56091=CARTESIAN_POINT ( 'NONE',  ( -110.7429703914275052, -295.7693060960082221, -293.4655916616991362 ) ) ;
#56092=CARTESIAN_POINT ( 'NONE',  ( -110.4136360351100308, -271.8502356476486170, -283.7365558647884427 ) ) ;
#56093=CARTESIAN_POINT ( 'NONE',  ( 26.52814733732099128, -273.6795811212947456, -228.2429407039788316 ) ) ;
#56094=CARTESIAN_POINT ( 'NONE',  ( -101.6086385096167959, -274.8096281454858740, -233.5464982536482239 ) ) ;
#56095=CARTESIAN_POINT ( 'NONE',  ( -38.91795226453715628, -293.1115901840395281, -197.0689526187062484 ) ) ;
#56097=CARTESIAN_POINT ( 'NONE',  ( -111.3619466279452297, -297.2377964174202134, -290.7037658316841657 ) ) ;
#56098=CARTESIAN_POINT ( 'NONE',  ( 21.22657140224840688, -288.6570643363683644, -314.0598147405129339 ) ) ;
#56099=CARTESIAN_POINT ( 'NONE',  ( -88.49030546875899006, -296.5503979021305554, -327.7733609191539585 ) ) ;
#56100=CARTESIAN_POINT ( 'NONE',  ( -65.57507530830704923, -295.9039270333842637, -341.9462958329617095 ) ) ;
#56101=CARTESIAN_POINT ( 'NONE',  ( 34.06801983643734388, -293.9195337676179065, -285.5753549825724349 ) ) ;
#56103=CARTESIAN_POINT ( 'NONE',  ( 21.61905308987663332, -276.8270026609069419, -223.0865746737032964 ) ) ;
#56105=CARTESIAN_POINT ( 'NONE',  ( -56.53523653229239443, -279.3189735065992636, -195.8002231839548983 ) ) ;
#56107=CARTESIAN_POINT ( 'NONE',  ( -1.344153737431386553, -277.5038249682741025, -334.1961303392545801 ) ) ;
#56108=CARTESIAN_POINT ( 'NONE',  ( 37.91741627755514799, -277.1793497440049237, -259.8711508077181520 ) ) ;
#56110=CARTESIAN_POINT ( 'NONE',  ( -70.86233746374362852, -275.5122971263422187, -337.8501813903125139 ) ) ;
#56111=CARTESIAN_POINT ( 'NONE',  ( -49.97968222912750491, -298.5380334163676253, -198.3599091295398011 ) ) ;
#56112=CARTESIAN_POINT ( 'NONE',  ( -96.08557286186945134, -294.5090240609454781, -314.7049276706690080 ) ) ;
#56114=CARTESIAN_POINT ( 'NONE',  ( -97.00269320569096010, -278.3918511870139127, -318.9625334014482405 ) ) ;
#56115=CARTESIAN_POINT ( 'NONE',  ( -66.80071543032686066, -277.6159260062093495, -337.1530817353018392 ) ) ;
#56117=CARTESIAN_POINT ( 'NONE',  ( -10.15344535591867547, -285.0844489322089430, -198.7917601921903952 ) ) ;
#56118=CARTESIAN_POINT ( 'NONE',  ( -51.48132906306179990, -299.8720352385096248, -196.4832810645096686 ) ) ;
#56120=CARTESIAN_POINT ( 'NONE',  ( 28.36831870069437400, -287.1840995813325890, -302.5293500126085178 ) ) ;
#56121=CARTESIAN_POINT ( 'NONE',  ( -34.24885224764852154, -278.3313906953229093, -196.3997135302541892 ) ) ;
#56122=CARTESIAN_POINT ( 'NONE',  ( -83.79575546704707278, -277.9749421671019718, -213.2215784465003594 ) ) ;
#56123=CARTESIAN_POINT ( 'NONE',  ( -108.3669899675573589, -282.3423169509645163, -292.6483879220964468 ) ) ;
#56124=CARTESIAN_POINT ( 'NONE',  ( -30.52643038339077819, -288.1383674637465901, -195.6200632462643512 ) ) ;
#56125=CARTESIAN_POINT ( 'NONE',  ( 19.49879119586512388, -277.4113360036536733, -316.8167879374884137 ) ) ;
#56127=CARTESIAN_POINT ( 'NONE',  ( -2.995052495117620506, -294.5060914721845506, -203.6735798760489615 ) ) ;
#56128=CARTESIAN_POINT ( 'NONE',  ( -42.75662538109197186, -275.3594626212182561, -346.1546045006214740 ) ) ;
#56129=CARTESIAN_POINT ( 'NONE',  ( -66.83619260384088534, -278.1005808026465616, -337.2488416847240273 ) ) ;
#56130=CARTESIAN_POINT ( 'NONE',  ( 12.48502450904744876, -284.3604744035619660, -326.7094229152319258 ) ) ;
#56132=CARTESIAN_POINT ( 'NONE',  ( 34.58464376219601633, -289.7689638375961181, -293.5109614464082028 ) ) ;
#56133=CARTESIAN_POINT ( 'NONE',  ( -58.69855347909871313, -293.3280512289803710, -342.3093950506277565 ) ) ;
#56135=CARTESIAN_POINT ( 'NONE',  ( -34.00162091959891342, -272.7798640336235394, -196.9439037219777333 ) ) ;
#56136=CARTESIAN_POINT ( 'NONE',  ( -14.44326268775513533, -290.4917740870004650, -199.7457723312913060 ) ) ;
#56139=CARTESIAN_POINT ( 'NONE',  ( -112.4858525041450719, -289.1994887688476865, -257.0922025289438579 ) ) ;
#56140=CARTESIAN_POINT ( 'NONE',  ( -94.02356840303724539, -285.4888981486163289, -317.6221614120665890 ) ) ;
#56141=CARTESIAN_POINT ( 'NONE',  ( 38.08186445193869929, -285.9143828498046673, -280.0169502407761684 ) ) ;
#56143=CARTESIAN_POINT ( 'NONE',  ( -49.53690538590971215, -287.3190342997609719, -197.7375001204646878 ) ) ;
#56144=CARTESIAN_POINT ( 'NONE',  ( -46.75575602308124701, -286.7325507428079732, -197.7569578035559630 ) ) ;
#56145=CARTESIAN_POINT ( 'NONE',  ( -112.3717159241940493, -292.6283266365251734, -262.8270252350141618 ) ) ;
#56146=CARTESIAN_POINT ( 'NONE',  ( 2.716951582430970902, -274.5995686634144590, -334.4899941275415927 ) ) ;
#56147=CARTESIAN_POINT ( 'NONE',  ( 35.18248142849234483, -276.2129943351353631, -296.3249920667107631 ) ) ;
#56148=CARTESIAN_POINT ( 'NONE',  ( -107.0294434081068431, -289.0105632392450730, -241.1561075897265027 ) ) ;
#56149=CARTESIAN_POINT ( 'NONE',  ( -37.12696551596004468, -277.0494984396683549, -347.3738772233279519 ) ) ;
#56150=CARTESIAN_POINT ( 'NONE',  ( -109.8918220812226281, -298.3048153400479237, -287.9741771711922524 ) ) ;
#56153=CARTESIAN_POINT ( 'NONE',  ( -110.7194928009815129, -283.3017751159325712, -265.4154428059761130 ) ) ;
#56154=CARTESIAN_POINT ( 'NONE',  ( -14.80384949957305984, -278.3438646973627897, -198.7731334203974711 ) ) ;
#56156=CARTESIAN_POINT ( 'NONE',  ( 38.24011964427000265, -273.8996157313088702, -259.8684408988631844 ) ) ;
#56157=CARTESIAN_POINT ( 'NONE',  ( -27.01530201320642988, -276.2659646161451974, -342.7300213178120885 ) ) ;
#56158=CARTESIAN_POINT ( 'NONE',  ( -6.456866650744444769, -296.1590791022027247, -337.2702714331201719 ) ) ;
#56159=CARTESIAN_POINT ( 'NONE',  ( -35.33030082650350323, -278.9971463005194323, -193.6835260780933083 ) ) ;
#56160=CARTESIAN_POINT ( 'NONE',  ( -53.18864949045561019, -296.2014857338569982, -341.9134967324556555 ) ) ;
#56161=CARTESIAN_POINT ( 'NONE',  ( -24.97094080966079588, -296.2128485230616661, -345.9149225143329431 ) ) ;
#56162=CARTESIAN_POINT ( 'NONE',  ( -91.84347862019282616, -297.0799420491071601, -221.7961496853052950 ) ) ;
#56163=CARTESIAN_POINT ( 'NONE',  ( -41.73477394707572330, -293.9970988171320414, -195.4386734662660388 ) ) ;
#56164=CARTESIAN_POINT ( 'NONE',  ( -80.93995271441103512, -285.6450764003434415, -206.8287161890721109 ) ) ;
#56165=CARTESIAN_POINT ( 'NONE',  ( 25.13956825401882966, -273.1167383573363168, -227.4849147633873940 ) ) ;
#56166=CARTESIAN_POINT ( 'NONE',  ( -4.334988585874142153, -288.4623828018427503, -339.9425218279787373 ) ) ;
#56167=CARTESIAN_POINT ( 'NONE',  ( -77.73260448470320227, -281.4872097975710972, -207.5267108538691616 ) ) ;
#56169=CARTESIAN_POINT ( 'NONE',  ( -93.42759532358584806, -284.2775400376325479, -223.2677977673970133 ) ) ;
#56170=CARTESIAN_POINT ( 'NONE',  ( -103.4065977414673654, -288.0807596467917620, -305.8636523889234127 ) ) ;
#56171=CARTESIAN_POINT ( 'NONE',  ( 30.52007695399996479, -26.23604800832216100, -343.5755449821854768 ) ) ;
#56172=CARTESIAN_POINT ( 'NONE',  ( -54.76494257819371825, -285.3298827151859314, -199.3551368336666201 ) ) ;
#56174=CARTESIAN_POINT ( 'NONE',  ( 6.799537257745960517, -283.4093464495015269, -333.2303568041374433 ) ) ;
#56175=CARTESIAN_POINT ( 'NONE',  ( -96.39017246408651829, -290.2727280257241773, -221.2888144382199300 ) ) ;
#56176=CARTESIAN_POINT ( 'NONE',  ( -98.79489647237402039, -280.7571348047457604, -225.2841770571867812 ) ) ;
#56177=CARTESIAN_POINT ( 'NONE',  ( -77.24966325893828412, -280.8444757689106837, -205.0261045969996587 ) ) ;
#56178=CARTESIAN_POINT ( 'NONE',  ( 31.35387658402771649, -281.7161544125552837, -295.2070776969027861 ) ) ;
#56179=CARTESIAN_POINT ( 'NONE',  ( 36.99967650147244314, -277.4249723052648164, -260.4434383497034560 ) ) ;
#56180=CARTESIAN_POINT ( 'NONE',  ( -90.71207447207180508, -295.7834944769748518, -325.9377074866476960 ) ) ;
#56181=CARTESIAN_POINT ( 'NONE',  ( -104.3324312289769296, -288.1359593528396772, -303.2866209571684522 ) ) ;
#56182=CARTESIAN_POINT ( 'NONE',  ( -104.2242475918841222, -295.0683892303916309, -300.5011037832608167 ) ) ;
#56185=CARTESIAN_POINT ( 'NONE',  ( 29.45379109670336604, -283.9103074744073751, -303.3366064260893609 ) ) ;
#56186=CARTESIAN_POINT ( 'NONE',  ( -110.2331408390485450, -296.2762403300752112, -266.0107895148270245 ) ) ;
#56187=CARTESIAN_POINT ( 'NONE',  ( 27.78256927198205162, -294.0987262493824801, -229.7599130250441988 ) ) ;
#56188=CARTESIAN_POINT ( 'NONE',  ( -93.49505205585893464, -284.5403364527106191, -317.1659653360856055 ) ) ;
#56190=CARTESIAN_POINT ( 'NONE',  ( 17.92853962991826933, -273.8785699404692764, -217.0117216562484259 ) ) ;
#56191=CARTESIAN_POINT ( 'NONE',  ( -42.05601121605359793, -292.6456027885760705, -193.6076942305612079 ) ) ;
#56192=CARTESIAN_POINT ( 'NONE',  ( -66.68839300440839679, -283.8113595802154805, -200.5107271523263819 ) ) ;
#56193=CARTESIAN_POINT ( 'NONE',  ( -111.5204605413089070, -290.6276088922380723, -290.9342994363199750 ) ) ;
#56194=CARTESIAN_POINT ( 'NONE',  ( 32.29247638116856933, -287.5936364837710357, -248.3381605330316972 ) ) ;
#56197=CARTESIAN_POINT ( 'NONE',  ( 160.6708272468242740, 217.8012694009499626, -202.3251110406953899 ) ) ;
#56198=CARTESIAN_POINT ( 'NONE',  ( -13.61894215047240664, -284.2697782174893177, -342.8865514901725078 ) ) ;
#56199=CARTESIAN_POINT ( 'NONE',  ( -54.42813229853333468, -283.3380690714491266, -195.3538533559490702 ) ) ;
#56201=CARTESIAN_POINT ( 'NONE',  ( 3.551296040237138740, -281.4084660206444255, -331.2664868571021657 ) ) ;
#56202=CARTESIAN_POINT ( 'NONE',  ( -7.896651663262564291, -276.3434994152810873, -341.5001718711064314 ) ) ;
#56203=CARTESIAN_POINT ( 'NONE',  ( -84.13375484440895491, -279.6968515543772469, -328.8275528808673016 ) ) ;
#56204=CARTESIAN_POINT ( 'NONE',  ( -92.65688847005533546, -240.4251198286245028, -339.9941278092445600 ) ) ;
#56205=CARTESIAN_POINT ( 'NONE',  ( 38.21490009151112588, -279.9789647599371278, -258.6241527485910865 ) ) ;
#56206=CARTESIAN_POINT ( 'NONE',  ( -88.81079852685080311, -283.3451212658792429, -216.2983885761691454 ) ) ;
#56207=CARTESIAN_POINT ( 'NONE',  ( -82.38812378547730475, -299.2071559892513051, -209.1010080315972459 ) ) ;
#56208=CARTESIAN_POINT ( 'NONE',  ( 34.38598553318960427, -294.2276716163444235, -284.2581518925622390 ) ) ;
#56210=CARTESIAN_POINT ( 'NONE',  ( -110.4618674326619328, -289.3338684781452912, -262.9662136043678515 ) ) ;
#56211=CARTESIAN_POINT ( 'NONE',  ( 39.52874431672737643, -276.1777548212208444, -268.3001577368727908 ) ) ;
#56212=CARTESIAN_POINT ( 'NONE',  ( -71.90772880776439990, -273.5820958407003900, -206.0071293961021297 ) ) ;
#56214=CARTESIAN_POINT ( 'NONE',  ( -46.82907625988709555, -272.8546930203463035, -194.2593295450973017 ) ) ;
#56219=CARTESIAN_POINT ( 'NONE',  ( -36.17487965774702730, -284.1168558368651702, -343.6609447530025250 ) ) ;
#56220=CARTESIAN_POINT ( 'NONE',  ( -94.21838698159886860, -281.0040325333411033, -219.9724634315274159 ) ) ;
#56221=CARTESIAN_POINT ( 'NONE',  ( -105.4371278660812123, -283.2498839915487565, -297.4514208470191079 ) ) ;
#56222=CARTESIAN_POINT ( 'NONE',  ( -38.39478520791233507, -281.8992335247962728, -196.1207729376543512 ) ) ;
#56223=CARTESIAN_POINT ( 'NONE',  ( 21.37776051075837458, -274.6519185729246146, -314.8890047105255690 ) ) ;
#56226=CARTESIAN_POINT ( 'NONE',  ( -71.48988190798968390, -278.2945715345014719, -339.1946890244837505 ) ) ;
#56230=CARTESIAN_POINT ( 'NONE',  ( -112.5646487503656630, -286.4647331273862960, -275.6284759522291097 ) ) ;
#56231=CARTESIAN_POINT ( 'NONE',  ( -4.751984350100819654, -291.6898812667785137, -204.8451606152623583 ) ) ;
#56232=CARTESIAN_POINT ( 'NONE',  ( -8.279354188717762852, -288.0300666213736349, -341.5701174569828140 ) ) ;
#56233=CARTESIAN_POINT ( 'NONE',  ( -101.8638743311186516, -283.2826316567292793, -233.9951015377691306 ) ) ;
#56234=CARTESIAN_POINT ( 'NONE',  ( -110.9801791004865237, -283.1198777690026418, -270.8956101083488193 ) ) ;
#56235=CARTESIAN_POINT ( 'NONE',  ( -96.59283317398147517, -288.1777366249448278, -314.7362757162314892 ) ) ;
#56236=CARTESIAN_POINT ( 'NONE',  ( 1.323459663542760900, -283.7285887856345994, -332.8074569326296910 ) ) ;
#56237=CARTESIAN_POINT ( 'NONE',  ( 4.727820773182989988, -274.4838739887581482, -332.4510210081800778 ) ) ;
#56239=CARTESIAN_POINT ( 'NONE',  ( 31.99266720023009114, -285.5422704550279036, -238.6241207358383463 ) ) ;
#56240=CARTESIAN_POINT ( 'NONE',  ( -26.59438322183623526, -300.1868440504003388, -195.3574452081263928 ) ) ;
#56241=CARTESIAN_POINT ( 'NONE',  ( -99.46653649144340648, -283.1247177515152771, -227.9545250757125814 ) ) ;
#56242=CIRCLE ( 'NONE', #45654, 1.000000000000000888 ) ;
#56243=CARTESIAN_POINT ( 'NONE',  ( -41.07512915030789458, -280.9452678741344585, -197.2210471851076932 ) ) ;
#56244=CARTESIAN_POINT ( 'NONE',  ( 29.77313388996562438, -289.1061269904064943, -236.5139987813681444 ) ) ;
#56247=CARTESIAN_POINT ( 'NONE',  ( -33.48344422893534045, -296.9241208876456994, -345.8354260878668356 ) ) ;
#56249=CARTESIAN_POINT ( 'NONE',  ( -105.1679627103966084, -276.9744033437324902, -238.2297838379603263 ) ) ;
#56250=CARTESIAN_POINT ( 'NONE',  ( -108.2142479086888045, -290.1277048480106373, -240.6754178707049618 ) ) ;
#56251=CARTESIAN_POINT ( 'NONE',  ( -38.37369884090015404, -293.4651714320732481, -344.1539048664077995 ) ) ;
#56252=CARTESIAN_POINT ( 'NONE',  ( -66.24834732509143009, -278.3504715100134490, -202.7778004026537246 ) ) ;
#56253=CARTESIAN_POINT ( 'NONE',  ( -109.9338283156847922, -270.8452343914886455, -253.8778802156916754 ) ) ;
#56254=CARTESIAN_POINT ( 'NONE',  ( 12.70285890476359469, -295.6520734641661647, -324.2526782947396100 ) ) ;
#56255=CARTESIAN_POINT ( 'NONE',  ( -85.33152481854862970, -299.9090924074130839, -210.2361428286348826 ) ) ;
#56256=CARTESIAN_POINT ( 'NONE',  ( -112.9681805602069744, -294.8988480238744501, -280.9146161741039691 ) ) ;
#56257=CARTESIAN_POINT ( 'NONE',  ( -23.61662371915925718, -290.4740980344088825, -342.9258863462990803 ) ) ;
#56258=CARTESIAN_POINT ( 'NONE',  ( -1.264941970054690001, -290.7639020069694311, -203.4848027728918680 ) ) ;
#56260=CARTESIAN_POINT ( 'NONE',  ( -79.88603296318224523, -292.8897146260090381, -210.2540428243744657 ) ) ;
#56262=CARTESIAN_POINT ( 'NONE',  ( -44.32577674786252686, -292.7645359449425086, -197.4828270622239756 ) ) ;
#56264=CARTESIAN_POINT ( 'NONE',  ( -111.9341454638480116, -291.9764053611519898, -252.9262156499200671 ) ) ;
#56265=CARTESIAN_POINT ( 'NONE',  ( 31.67678337766244923, -279.1781233808102343, -240.1145357874084709 ) ) ;
#56266=CARTESIAN_POINT ( 'NONE',  ( 2.240500172301783000, -292.5982639183745846, -208.9640595639771448 ) ) ;
#56267=CARTESIAN_POINT ( 'NONE',  ( -42.43005377325469851, -279.9896423994456995, -193.5294275340110346 ) ) ;
#56268=CARTESIAN_POINT ( 'NONE',  ( -30.22107432238242808, -282.6311090432532751, -347.0099338875499484 ) ) ;
#56269=CARTESIAN_POINT ( 'NONE',  ( -97.25096915064618486, -287.9377561655864497, -315.2256598190316481 ) ) ;
#56270=CARTESIAN_POINT ( 'NONE',  ( 27.54986949932021290, -279.2070033484595228, -234.3063031964529159 ) ) ;
#56271=CARTESIAN_POINT ( 'NONE',  ( -79.78485323236849069, -283.4785847621789117, -208.4633460878366975 ) ) ;
#56272=CARTESIAN_POINT ( 'NONE',  ( 82.64890176555634582, -299.5541904835127980, -192.9639945212225882 ) ) ;
#56273=CARTESIAN_POINT ( 'NONE',  ( 12.55356583895141220, -279.2129172431603479, -212.6275039862651965 ) ) ;
#56274=CARTESIAN_POINT ( 'NONE',  ( 20.06454712660518780, -285.7801732321295844, -219.4298294336416859 ) ) ;
#56276=CARTESIAN_POINT ( 'NONE',  ( -3.284999187389276543, -294.1099210363839802, -204.8891274986903568 ) ) ;
#56277=CARTESIAN_POINT ( 'NONE',  ( 2.098208443403834167, -275.9946387408119222, -204.9157216251434477 ) ) ;
#56278=CARTESIAN_POINT ( 'NONE',  ( -107.8417834087898086, -277.9676861758980522, -289.3828356823390777 ) ) ;
#56279=CARTESIAN_POINT ( 'NONE',  ( -112.9253662689182818, -290.9035425593309014, -255.5917613736295948 ) ) ;
#56280=CARTESIAN_POINT ( 'NONE',  ( -68.61324321467263587, -281.5397302433052573, -339.1604726839812542 ) ) ;
#56281=CARTESIAN_POINT ( 'NONE',  ( -108.9380767348257422, -289.8134852999838813, -254.9543887493984755 ) ) ;
#56282=CARTESIAN_POINT ( 'NONE',  ( -89.34418774903762994, -293.7836561763161285, -324.4765332201062051 ) ) ;
#56285=CARTESIAN_POINT ( 'NONE',  ( -33.49893427736539309, -291.6094427673351106, -197.3882041903070785 ) ) ;
#56287=CARTESIAN_POINT ( 'NONE',  ( -67.74223827176244583, -300.1233781216987495, -207.3071070584150277 ) ) ;
#56288=CARTESIAN_POINT ( 'NONE',  ( -105.7534716745016965, -295.1597832577228928, -305.3013691916552261 ) ) ;
#56289=CARTESIAN_POINT ( 'NONE',  ( 32.41920201379472388, -280.0756181050880400, -300.0537876351163504 ) ) ;
#56290=CARTESIAN_POINT ( 'NONE',  ( -112.6485215791210379, -285.6937724263038945, -284.1490872394634835 ) ) ;
#56291=CARTESIAN_POINT ( 'NONE',  ( 35.45172209074848979, -287.4662348023951495, -276.4834481234726127 ) ) ;
#56292=CARTESIAN_POINT ( 'NONE',  ( 24.57736227788190675, -277.6213489690156280, -310.4144435115568399 ) ) ;
#56293=CARTESIAN_POINT ( 'NONE',  ( -110.3834894310941621, -294.7715376765541464, -254.9132797313550327 ) ) ;
#56294=CARTESIAN_POINT ( 'NONE',  ( -58.67924790920642408, -297.0920617900294474, -341.2320081014541415 ) ) ;
#56295=CARTESIAN_POINT ( 'NONE',  ( -76.58099912719606550, -276.3845421949446859, -332.4483759141702990 ) ) ;
#56298=CARTESIAN_POINT ( 'NONE',  ( -94.63867754377160679, -295.5210027576895300, -321.7889354388340735 ) ) ;
#56299=CARTESIAN_POINT ( 'NONE',  ( 37.09534282965131524, -289.4809019409074153, -271.0250687287473852 ) ) ;
#56300=CARTESIAN_POINT ( 'NONE',  ( 82.17440492340898572, -297.5479941798179766, -195.4018648718562758 ) ) ;
#56301=CARTESIAN_POINT ( 'NONE',  ( 34.62349548100537078, -288.3727319458883471, -283.2025855520745381 ) ) ;
#56303=CARTESIAN_POINT ( 'NONE',  ( -33.91374910648440988, -279.1530423493786088, -193.6729874459910548 ) ) ;
#56304=CARTESIAN_POINT ( 'NONE',  ( -94.57016159653069565, -296.5055381387020930, -321.7443005989644575 ) ) ;
#56305=CARTESIAN_POINT ( 'NONE',  ( -85.70604012864082222, -289.5309752984884994, -211.9732409193950389 ) ) ;
#56306=CARTESIAN_POINT ( 'NONE',  ( -114.1000937285443513, -296.9665543338628595, -263.8764648965195647 ) ) ;
#56308=CARTESIAN_POINT ( 'NONE',  ( 30.84662000572555129, -293.5366409679363073, -244.2375561265371857 ) ) ;
#56313=CARTESIAN_POINT ( 'NONE',  ( 11.98253380504862520, -289.9008660174117722, -328.5833448195132860 ) ) ;
#56314=CARTESIAN_POINT ( 'NONE',  ( -19.11405058567862625, -282.7662352645559167, -190.3538533559490702 ) ) ;
#56316=CARTESIAN_POINT ( 'NONE',  ( 29.66899579363884598, -281.3920319619346628, -308.1906945360046848 ) ) ;
#56317=CARTESIAN_POINT ( 'NONE',  ( -23.70708394855249068, -284.8776729340844440, -343.9418604719035670 ) ) ;
#56318=CARTESIAN_POINT ( 'NONE',  ( 38.75896854923772850, -286.2135528554616144, -277.2382190204973540 ) ) ;
#56320=CARTESIAN_POINT ( 'NONE',  ( -102.9231427508413788, -288.1597575417061421, -305.6896235641398789 ) ) ;
#56321=CARTESIAN_POINT ( 'NONE',  ( 37.00207179470736207, -277.2269286007979190, -255.7560141021987761 ) ) ;
#56324=CARTESIAN_POINT ( 'NONE',  ( -70.45280026804331897, -277.5014054036172411, -335.4199763150070339 ) ) ;
#56325=CARTESIAN_POINT ( 'NONE',  ( -1.909417204406070878, -279.8833477539669161, -206.4201608802100623 ) ) ;
#56326=CARTESIAN_POINT ( 'NONE',  ( -11.95548255968575191, -277.8091189405590171, -342.7841683369392740 ) ) ;
#56327=CARTESIAN_POINT ( 'NONE',  ( -113.3212225893833818, -277.4747514743254442, -260.2052129746995206 ) ) ;
#56328=CARTESIAN_POINT ( 'NONE',  ( -112.1726278936763492, -268.3392834764117652, -295.5492975640193549 ) ) ;
#56329=CARTESIAN_POINT ( 'NONE',  ( -101.0200949150615912, -274.0609840243497501, -227.3959344430673752 ) ) ;
#56331=CARTESIAN_POINT ( 'NONE',  ( -65.34311428139507427, -299.1186235670851943, -199.2093613379682040 ) ) ;
#56332=CARTESIAN_POINT ( 'NONE',  ( -4.771743288812468897, -291.1233781216987495, -337.9199732462171255 ) ) ;
#56334=CARTESIAN_POINT ( 'NONE',  ( 35.06669393023508974, -288.7833723934188583, -281.8976726960947872 ) ) ;
#56335=CARTESIAN_POINT ( 'NONE',  ( -80.38292546119866699, -287.2382810150907630, -207.6762968376524157 ) ) ;
#56336=CARTESIAN_POINT ( 'NONE',  ( 34.66926882740423110, -286.7312232153552145, -257.4931494000165912 ) ) ;
#56337=CARTESIAN_POINT ( 'NONE',  ( -70.44932511048989454, -282.9845510535215567, -339.8263573073675161 ) ) ;
#56338=CARTESIAN_POINT ( 'NONE',  ( -16.67841166895991378, -278.7234554548429060, -199.5129075359699868 ) ) ;
#56339=CARTESIAN_POINT ( 'NONE',  ( -77.74080598953176491, -287.3642007066288784, -208.0202818289762376 ) ) ;
#56340=CARTESIAN_POINT ( 'NONE',  ( -2.807201313430653933, -278.9971878765248903, -205.2462958701118794 ) ) ;
#56341=CARTESIAN_POINT ( 'NONE',  ( -87.41940843683433116, -279.0837538562848295, -324.1520708242007913 ) ) ;
#56342=CARTESIAN_POINT ( 'NONE',  ( 11.79372153771742227, -276.8402246400063405, -324.5010119735229068 ) ) ;
#56343=CARTESIAN_POINT ( 'NONE',  ( 22.08732485151113423, -286.9991296965905008, -318.7160061877781345 ) ) ;
#56344=CARTESIAN_POINT ( 'NONE',  ( -81.46046194946160313, -284.4380496721336158, -333.3360457249852971 ) ) ;
#56345=CARTESIAN_POINT ( 'NONE',  ( -114.1464828408261241, -284.9774276322870605, -275.7197462586422603 ) ) ;
#56346=CARTESIAN_POINT ( 'NONE',  ( 31.06955988498283006, -281.3773405714608771, -244.7426012350530868 ) ) ;
#56350=CARTESIAN_POINT ( 'NONE',  ( -89.94566032384366849, -293.1796539632111376, -215.7618773006412880 ) ) ;
#56351=CARTESIAN_POINT ( 'NONE',  ( -58.78432046757862395, -290.4652603212256849, -196.9205821417289997 ) ) ;
#56352=CARTESIAN_POINT ( 'NONE',  ( -103.4122115735392100, -272.0367976005389323, -238.7684611663970315 ) ) ;
#56353=CARTESIAN_POINT ( 'NONE',  ( 39.39981045361309953, -292.9718554279172054, -276.0398927534272389 ) ) ;
#56354=CARTESIAN_POINT ( 'NONE',  ( -110.3847005139535042, -289.1646141710455709, -260.2146500376612153 ) ) ;
#56355=CARTESIAN_POINT ( 'NONE',  ( 26.65781588813821301, -292.2950747541514716, -307.5368622444860875 ) ) ;
#56356=CARTESIAN_POINT ( 'NONE',  ( -92.70116429069648234, -291.0731096436051644, -318.6289601620851499 ) ) ;
#56358=CARTESIAN_POINT ( 'NONE',  ( -95.71691776013170738, -291.9039756178406719, -317.4699461381828201 ) ) ;
#56359=CARTESIAN_POINT ( 'NONE',  ( -109.4656954231785306, -288.8240063700159226, -249.1913817905198130 ) ) ;
#56361=CARTESIAN_POINT ( 'NONE',  ( -111.0088617772822630, -292.7339166449121421, -256.2172616351275565 ) ) ;
#56362=CARTESIAN_POINT ( 'NONE',  ( 2.565225255155341610, -287.5430868522681180, -208.9539054237454536 ) ) ;
#56363=CARTESIAN_POINT ( 'NONE',  ( 36.26138935328503976, -295.3561070711276102, -255.0464579060937069 ) ) ;
#56366=CARTESIAN_POINT ( 'NONE',  ( -27.24246546777073519, -276.1596564890069772, -195.6334513602025993 ) ) ;
#56367=CARTESIAN_POINT ( 'NONE',  ( -105.8184513689372466, -295.2981803934353593, -305.3365452077952682 ) ) ;
#56368=CARTESIAN_POINT ( 'NONE',  ( -2.415952884151053581, -272.7607832837292108, -205.1064921343491108 ) ) ;
#56369=CARTESIAN_POINT ( 'NONE',  ( -109.2169069403395554, -276.3810697804223651, -289.7329750374756259 ) ) ;
#56370=CARTESIAN_POINT ( 'NONE',  ( -93.22603672602734548, -274.4305195931991079, -222.7594525282359541 ) ) ;
#56371=CARTESIAN_POINT ( 'NONE',  ( -110.6848704805083372, -297.8909408968103776, -276.9704801140501900 ) ) ;
#56373=CARTESIAN_POINT ( 'NONE',  ( -95.42348713590395448, -297.9796698452749979, -225.8535378633549442 ) ) ;
#56376=CARTESIAN_POINT ( 'NONE',  ( 17.17926379417045624, -284.8447838605778202, -218.2678467999553789 ) ) ;
#56377=CARTESIAN_POINT ( 'NONE',  ( -97.84200078662045996, -272.9543443512566796, -229.4210500452513486 ) ) ;
#56379=CARTESIAN_POINT ( 'NONE',  ( 24.70327030290053116, -286.9464343003230624, -224.7604420641200704 ) ) ;
#56380=CARTESIAN_POINT ( 'NONE',  ( -100.6656204782153168, -289.6406795300139265, -314.1312608087405920 ) ) ;
#56381=CARTESIAN_POINT ( 'NONE',  ( -108.3104668044043564, -298.8588096818442637, -245.0265377043011767 ) ) ;
#56382=CARTESIAN_POINT ( 'NONE',  ( 34.50333385887570614, -291.8226894927343551, -291.3432020639249913 ) ) ;
#56383=ADVANCED_FACE ( 'NONE', ( #38900 ), #45511, .F. ) ;
#56384=AXIS2_PLACEMENT_3D ( 'NONE', #37482, #44119, #10001 ) ;
#56385=CARTESIAN_POINT ( 'NONE',  ( 36.02457618131488459, -280.4618263272919876, -247.5236855309644000 ) ) ;
#56387=CARTESIAN_POINT ( 'NONE',  ( 10.59707575819633618, -291.9094976428776249, -330.5268031993606428 ) ) ;
#56390=CARTESIAN_POINT ( 'NONE',  ( 16.29067623551082633, -287.0645619213318582, -320.5423392063346455 ) ) ;
#56392=CARTESIAN_POINT ( 'NONE',  ( -51.14385109387259121, -287.2282702336642046, -344.1332859679654916 ) ) ;
#56393=CARTESIAN_POINT ( 'NONE',  ( -92.55030523426522393, -274.7630793605416670, -221.5480287987056442 ) ) ;
#56394=CARTESIAN_POINT ( 'NONE',  ( 28.76763901231315756, -282.4752722187291170, -232.0445214468282416 ) ) ;
#56395=CARTESIAN_POINT ( 'NONE',  ( -106.2583369648586284, -294.9711037820858905, -239.7542778171975897 ) ) ;
#56396=CARTESIAN_POINT ( 'NONE',  ( 7.793960597335130913, -282.4162055343190900, -327.7996435053851769 ) ) ;
#56397=CARTESIAN_POINT ( 'NONE',  ( -104.6018702781830569, -296.2316398208089367, -307.9543686941682950 ) ) ;
#56398=CARTESIAN_POINT ( 'NONE',  ( -75.58686874495387542, -299.0523962641618709, -207.3097658321668462 ) ) ;
#56399=CARTESIAN_POINT ( 'NONE',  ( 37.24936808194060944, -285.7897704759747626, -282.7403791609850146 ) ) ;
#56400=CARTESIAN_POINT ( 'NONE',  ( 36.89534189518388274, -283.6893232533773812, -281.0317431091017966 ) ) ;
#56401=CARTESIAN_POINT ( 'NONE',  ( -109.2745235932589765, -295.7925843850696879, -256.5438441849921105 ) ) ;
#56403=DIRECTION ( 'NONE',  ( -1.000000000000000000, -0.000000000000000000, -0.000000000000000000 ) ) ;
#56404=CARTESIAN_POINT ( 'NONE',  ( -67.19474045159624609, -285.4253656885182977, -338.7902156312812849 ) ) ;
#56406=CARTESIAN_POINT ( 'NONE',  ( -95.99890600148557951, -293.4094976428775681, -317.0979686699210447 ) ) ;
#56407=CARTESIAN_POINT ( 'NONE',  ( 37.74569222420570469, -274.9545116771682274, -286.7333592771032045 ) ) ;
#56408=CARTESIAN_POINT ( 'NONE',  ( 29.85657639541818398, -293.0010133415241853, -241.7117630421124090 ) ) ;
#56409=CARTESIAN_POINT ( 'NONE',  ( 34.32895408557164529, -283.2970485482736080, -287.5620208184632247 ) ) ;
#56410=CARTESIAN_POINT ( 'NONE',  ( 5.881650902148037652, -278.0556472069850429, -330.2421458938829346 ) ) ;
#56412=CARTESIAN_POINT ( 'NONE',  ( -105.2520809208994450, -285.5211805215334380, -305.5020222564936603 ) ) ;
#56413=CARTESIAN_POINT ( 'NONE',  ( -107.3692767163192485, -283.0572798969670316, -292.3444985727988978 ) ) ;
#56414=CARTESIAN_POINT ( 'NONE',  ( -104.9224074670407560, -280.1225945586293733, -303.0057886147212116 ) ) ;
#56415=CARTESIAN_POINT ( 'NONE',  ( 36.58525964960605137, -275.4466457618862023, -248.6386858202942562 ) ) ;
#56416=CARTESIAN_POINT ( 'NONE',  ( 39.31752326143391230, -275.2881896637475165, -262.5824542022432411 ) ) ;
#56417=CARTESIAN_POINT ( 'NONE',  ( -15.14049336077824215, -296.6827114616025938, -341.4675825952333525 ) ) ;
#56420=CARTESIAN_POINT ( 'NONE',  ( -111.9190304113460854, -294.8615671220086369, -256.9997075063920988 ) ) ;
#56421=CARTESIAN_POINT ( 'NONE',  ( -13.77147239918030586, -276.2456213985070121, -339.5694344242997431 ) ) ;
#56422=CARTESIAN_POINT ( 'NONE',  ( 32.78708948229623843, -295.4603535007067308, -300.5722172756474606 ) ) ;
#56423=CARTESIAN_POINT ( 'NONE',  ( 38.21718242986301561, -294.9166731736594329, -283.0448169870533661 ) ) ;
#56424=CARTESIAN_POINT ( 'NONE',  ( -111.0877877734702821, -292.7196854543867630, -257.3547263124657434 ) ) ;
#56425=CARTESIAN_POINT ( 'NONE',  ( -110.9304309794785013, -276.7268931438641744, -256.7696824266112117 ) ) ;
#56426=CARTESIAN_POINT ( 'NONE',  ( -86.45218274701142036, -281.2839572177943523, -214.4194099985491846 ) ) ;
#56427=CARTESIAN_POINT ( 'NONE',  ( -89.52847982924940595, -293.8739317488976326, -323.5170472912803916 ) ) ;
#56428=CARTESIAN_POINT ( 'NONE',  ( 38.38597053036861695, -283.4427150067806451, -272.7329051855021476 ) ) ;
#56429=CARTESIAN_POINT ( 'NONE',  ( -72.51027266384272707, -284.4953637003557674, -206.0242369529304085 ) ) ;
#56430=CARTESIAN_POINT ( 'NONE',  ( -111.2916113504647768, -274.2541639013562076, -270.3827886689474553 ) ) ;
#56431=CARTESIAN_POINT ( 'NONE',  ( -65.09732603224448155, -285.3460844923644686, -202.7668437869050990 ) ) ;
#56433=CARTESIAN_POINT ( 'NONE',  ( 32.11828435561940864, -283.0511563316167098, -302.9947871730552151 ) ) ;
#56435=CARTESIAN_POINT ( 'NONE',  ( -113.5106799047506456, -283.2447218810432901, -278.5033067414787524 ) ) ;
#56436=CARTESIAN_POINT ( 'NONE',  ( -113.8106557013271072, -279.5851393093995512, -263.0482996926588726 ) ) ;
#56437=CARTESIAN_POINT ( 'NONE',  ( -90.82911165092819772, -279.3140722481486478, -324.8575574266139938 ) ) ;
#56438=CARTESIAN_POINT ( 'NONE',  ( -25.41958609695204885, -280.8517118272686730, -194.3928615634703476 ) ) ;
#56440=CARTESIAN_POINT ( 'NONE',  ( -102.0455923789670294, -299.4805209788416391, -239.2376011013261916 ) ) ;
#56441=CARTESIAN_POINT ( 'NONE',  ( 195.2426427160663991, 278.4661148582146097, -125.8609867272279246 ) ) ;
#56442=EDGE_LOOP ( 'NONE', ( #13836, #39372, #18623, #2026 ) ) ;
#56444=CARTESIAN_POINT ( 'NONE',  ( -69.08280927211342259, -275.6339466775700657, -202.5788634308241001 ) ) ;
#56445=CARTESIAN_POINT ( 'NONE',  ( 153.0615653321293905, 207.2999644492867048, -217.0734274107136628 ) ) ;
#56447=CARTESIAN_POINT ( 'NONE',  ( -4.819586325188885745, -278.5027187778517259, -203.1736271744400710 ) ) ;
#56448=CARTESIAN_POINT ( 'NONE',  ( -8.911432685590609637, -294.1791215237471988, -199.8934381040679398 ) ) ;
#56449=CARTESIAN_POINT ( 'NONE',  ( 34.58495855550241060, -292.7278342509392814, -257.2358790163861499 ) ) ;
#56450=CARTESIAN_POINT ( 'NONE',  ( -95.41597551512251130, -289.3771266694707833, -320.8279926791381627 ) ) ;
#56452=CARTESIAN_POINT ( 'NONE',  ( 0.2348002737982404775, -293.1366900232138732, -336.9089753550182991 ) ) ;
#56453=CARTESIAN_POINT ( 'NONE',  ( -38.61853276064386620, -284.4357829947898040, -196.5595426480916217 ) ) ;
#56454=CARTESIAN_POINT ( 'NONE',  ( -102.2144349037427702, -292.8990378016016507, -234.1667847760658674 ) ) ;
#56455=CARTESIAN_POINT ( 'NONE',  ( -109.4602149205049528, -285.6819473107316298, -284.5090260726261704 ) ) ;
#56457=CARTESIAN_POINT ( 'NONE',  ( -53.35198213959034774, -292.7930332494909180, -195.2302170355795283 ) ) ;
#56459=CARTESIAN_POINT ( 'NONE',  ( -36.18627523469005780, -283.5296266779871530, -343.4135199634243349 ) ) ;
#56460=CARTESIAN_POINT ( 'NONE',  ( 21.05494722386966799, -293.0188515772367168, -319.9377283723553660 ) ) ;
#56461=CARTESIAN_POINT ( 'NONE',  ( 23.16664006803374676, -288.9895226902963259, -317.7415681150929458 ) ) ;
#56463=CARTESIAN_POINT ( 'NONE',  ( -97.23821350659802931, -290.3964065975628159, -318.6720014105655423 ) ) ;
#56464=CARTESIAN_POINT ( 'NONE',  ( 21.17475724337224818, -288.3314498388709239, -314.0263356679111553 ) ) ;
#56467=CARTESIAN_POINT ( 'NONE',  ( -110.4368107183282319, -298.6685435892064788, -250.2318759761165268 ) ) ;
#56469=CARTESIAN_POINT ( 'NONE',  ( -34.76316277018695899, -296.7686317458075109, -193.8548274820176971 ) ) ;
#56470=CARTESIAN_POINT ( 'NONE',  ( -7.893869019877665316, -279.5064529411663443, -203.2934392616369905 ) ) ;
#56471=CARTESIAN_POINT ( 'NONE',  ( -68.81315215092013204, -273.1570677097084854, -200.1393663240377236 ) ) ;
#56472=CARTESIAN_POINT ( 'NONE',  ( -23.40652372552063909, -293.3507748869216130, -342.7770037375145762 ) ) ;
#56473=CARTESIAN_POINT ( 'NONE',  ( 12.20852345766576086, -276.5126371984072193, -215.3125929431929251 ) ) ;
#56474=CARTESIAN_POINT ( 'NONE',  ( -33.72794539926945134, -296.3378518967315927, -196.3488791081413183 ) ) ;
#56475=CARTESIAN_POINT ( 'NONE',  ( -15.45989597189430675, -295.9677482840294260, -340.4739651587536855 ) ) ;
#56476=CARTESIAN_POINT ( 'NONE',  ( -78.11027596536193585, -296.6938778292721963, -331.3498351730605691 ) ) ;
#56478=CARTESIAN_POINT ( 'NONE',  ( -50.31110161546963866, -296.8150499799922954, -345.5026824115543036 ) ) ;
#56480=CARTESIAN_POINT ( 'NONE',  ( -95.90164498658693049, -295.1990049693231413, -223.2361639816649301 ) ) ;
#56481=CARTESIAN_POINT ( 'NONE',  ( -9.696609853111157307, -293.0743696447640332, -202.6342113768496915 ) ) ;
#56482=CARTESIAN_POINT ( 'NONE',  ( -87.93774596085788176, -274.1687926498977390, -212.4613197160124116 ) ) ;
#56483=CARTESIAN_POINT ( 'NONE',  ( -88.32584239325321107, -289.8959332430033555, -217.2247908743093490 ) ) ;
#56484=CARTESIAN_POINT ( 'NONE',  ( -38.12820669670584550, -276.0424522993371284, -195.3652376922328244 ) ) ;
#56485=CARTESIAN_POINT ( 'NONE',  ( -105.5572855983578933, -273.5051798885942844, -234.6627992068795834 ) ) ;
#56486=CARTESIAN_POINT ( 'NONE',  ( -93.63258947546353284, -297.5447957752236903, -223.8290509811140510 ) ) ;
#56488=CARTESIAN_POINT ( 'NONE',  ( -28.44476837229287725, -282.1442415856832326, -195.4804942847801783 ) ) ;
#56489=CARTESIAN_POINT ( 'NONE',  ( 19.77177666151919055, -279.5422357415955616, -219.4361193334763414 ) ) ;
#56491=CARTESIAN_POINT ( 'NONE',  ( -89.14956780075755205, -277.1071420590648700, -327.1876754494122110 ) ) ;
#56492=CARTESIAN_POINT ( 'NONE',  ( 37.20630972042400231, -279.7518070603735509, -254.5177861087676376 ) ) ;
#56493=CARTESIAN_POINT ( 'NONE',  ( 5.850221493657672411, -280.4684074958502151, -331.9429301148162494 ) ) ;
#56494=CARTESIAN_POINT ( 'NONE',  ( -66.02621890771744972, -272.2439711651368839, -202.5925906230976352 ) ) ;
#56495=CARTESIAN_POINT ( 'NONE',  ( -54.22143493831853789, -279.2689642414715649, -343.4896148003367671 ) ) ;
#56498=CARTESIAN_POINT ( 'NONE',  ( -96.54257871092923438, -295.4389853515199320, -222.7246824237597593 ) ) ;
#56499=CARTESIAN_POINT ( 'NONE',  ( -5.280555885609304667, -290.4920756620618363, -202.1666179325429482 ) ) ;
#56500=CARTESIAN_POINT ( 'NONE',  ( -86.51303194554405707, -291.3910918651312727, -211.0366747779846150 ) ) ;
#56501=CARTESIAN_POINT ( 'NONE',  ( 36.92842868515545263, -277.7047962698657670, -282.2633088143482496 ) ) ;
#56502=CARTESIAN_POINT ( 'NONE',  ( -43.62496007597515302, -271.9727322638058808, -195.5726732523458509 ) ) ;
#56505=CARTESIAN_POINT ( 'NONE',  ( -35.90165130381072345, -284.9544062847471650, -345.9202695840223782 ) ) ;
#56507=CARTESIAN_POINT ( 'NONE',  ( -24.98171654488527338, -284.2094912620926834, -196.3347462400582515 ) ) ;
#56508=CARTESIAN_POINT ( 'NONE',  ( -12.89035065966967508, -293.5222210471893050, -339.6191550207059322 ) ) ;
#56509=CARTESIAN_POINT ( 'NONE',  ( 35.20812380990154367, -285.4877021766924940, -254.6325284008937899 ) ) ;
#56511=CARTESIAN_POINT ( 'NONE',  ( -25.92748607628257318, -292.9066093403312721, -344.4874720277475717 ) ) ;
#56512=CARTESIAN_POINT ( 'NONE',  ( -97.50978271558163613, -282.3993071669198116, -317.2920203087631990 ) ) ;
#56513=CARTESIAN_POINT ( 'NONE',  ( -66.40329534439872816, -281.2653028192255533, -202.5102867880562485 ) ) ;
#56514=CARTESIAN_POINT ( 'NONE',  ( -102.1905362386951737, -286.2939159587666609, -229.5856698161211682 ) ) ;
#56515=CARTESIAN_POINT ( 'NONE',  ( 36.35402916168109755, -279.5572344014840951, -251.8431942062244104 ) ) ;
#56516=CARTESIAN_POINT ( 'NONE',  ( 17.77618855459306957, -286.8697964585653040, -222.4965345500855278 ) ) ;
#56517=CIRCLE ( 'NONE', #20195, 2.397123461337413719 ) ;
#56518=CARTESIAN_POINT ( 'NONE',  ( -110.5542632014368820, -280.0811463999183388, -262.4354489847819991 ) ) ;
#56519=CARTESIAN_POINT ( 'NONE',  ( -95.39492501369525712, -278.7299412020260547, -314.8855473203295787 ) ) ;
#56520=CARTESIAN_POINT ( 'NONE',  ( -72.86051582443228369, -287.5642994051705728, -203.8441525607969425 ) ) ;
#56522=EDGE_LOOP ( 'NONE', ( #22634, #47781 ) ) ;
#56524=CARTESIAN_POINT ( 'NONE',  ( -62.84304624642552994, -297.5624462130562051, -197.7065837080185418 ) ) ;
#56525=CARTESIAN_POINT ( 'NONE',  ( 4.558267796475975686, -290.4639752367180563, -332.1991768912891985 ) ) ;
#56527=CARTESIAN_POINT ( 'NONE',  ( 35.59421657381088266, -301.4082689599840705, -190.3320873922940848 ) ) ;
#56529=CARTESIAN_POINT ( 'NONE',  ( -27.21761594896082670, -272.1802448863628570, -195.8272071098441245 ) ) ;
#56530=CARTESIAN_POINT ( 'NONE',  ( 36.31459455635539513, -291.7044576063424870, -250.7866194261436021 ) ) ;
#56531=CARTESIAN_POINT ( 'NONE',  ( -110.4436330666481183, -271.9008437819409210, -270.3528433432777547 ) ) ;
#56533=CARTESIAN_POINT ( 'NONE',  ( -80.80092267947240714, -291.1737327556389232, -329.9393408022421568 ) ) ;
#56534=CARTESIAN_POINT ( 'NONE',  ( -27.44476216906243593, -281.9396152701979190, -196.9605669658214140 ) ) ;
#56535=CARTESIAN_POINT ( 'NONE',  ( -37.48214759217880498, -290.4791072874975839, -346.7847344300932946 ) ) ;
#56536=CARTESIAN_POINT ( 'NONE',  ( -103.3643333324506983, -291.3597523499364570, -309.1221744869474719 ) ) ;
#56537=CARTESIAN_POINT ( 'NONE',  ( -16.64372211822849579, -288.3195797906191160, -198.2194200888332034 ) ) ;
#56538=CARTESIAN_POINT ( 'NONE',  ( 12.99056856368130042, -280.8994477234854230, -212.0888026619383595 ) ) ;
#56539=CARTESIAN_POINT ( 'NONE',  ( -41.88390723272224392, -293.1886797296315308, -345.8358864541437470 ) ) ;
#56540=CARTESIAN_POINT ( 'NONE',  ( 1.375809934639267373, -280.3874398222892523, -203.7425091662561556 ) ) ;
#56542=CARTESIAN_POINT ( 'NONE',  ( 27.86284381676375688, -277.8901445823409517, -305.9543124942162535 ) ) ;
#56544=CARTESIAN_POINT ( 'NONE',  ( -54.42813229853333468, -297.7662352645559167, -345.3683826091709648 ) ) ;
#56545=CARTESIAN_POINT ( 'NONE',  ( 35.51540069524032361, -274.0669267218495975, -291.9897697811916260 ) ) ;
#56546=CARTESIAN_POINT ( 'NONE',  ( 33.01701867748859343, -281.3198119650901958, -290.0496712513210014 ) ) ;
#56548=CARTESIAN_POINT ( 'NONE',  ( -62.26223509124600497, -278.5741516955810653, -342.8531424128390768 ) ) ;
#56549=CARTESIAN_POINT ( 'NONE',  ( -69.72323517981750740, -274.9317332416228510, -204.3862768131380108 ) ) ;
#56550=CARTESIAN_POINT ( 'NONE',  ( -99.14764263528250865, -284.2186387920868924, -224.7451580521282324 ) ) ;
#56551=CARTESIAN_POINT ( 'NONE',  ( -111.3180478612490987, -292.2652082137114462, -273.9805566028367707 ) ) ;
#56552=CARTESIAN_POINT ( 'NONE',  ( -109.3525769114165058, -274.4697063331597064, -245.4437738324730276 ) ) ;
#56554=CARTESIAN_POINT ( 'NONE',  ( -87.72428621854042774, -274.6810516230699477, -212.7155593108392679 ) ) ;
#56556=CARTESIAN_POINT ( 'NONE',  ( -107.5341244964257754, -298.8914970360070242, -244.2682663688783578 ) ) ;
#56557=CARTESIAN_POINT ( 'NONE',  ( -96.58302693451905441, -281.9238446275705314, -316.1039603026502505 ) ) ;
#56558=CARTESIAN_POINT ( 'NONE',  ( -103.1955543923324967, -290.7404473726354581, -230.3959139943439993 ) ) ;
#56559=CARTESIAN_POINT ( 'NONE',  ( 37.23162044898293743, -273.5168815500396704, -266.0689725091951345 ) ) ;
#56560=CARTESIAN_POINT ( 'NONE',  ( 11.91438134250634029, -289.9808595601708703, -328.5012835449879844 ) ) ;
#56562=CARTESIAN_POINT ( 'NONE',  ( -104.9829945871630770, -289.8516009614157838, -241.9645871083978648 ) ) ;
#56563=VERTEX_POINT ( 'NONE', #53114 ) ;
#56564=CARTESIAN_POINT ( 'NONE',  ( -113.7789321490720056, -289.1522021094442039, -268.3519541098652326 ) ) ;
#56565=CARTESIAN_POINT ( 'NONE',  ( -98.13062750240479204, -289.6571539803717883, -310.8411915928285794 ) ) ;
#56566=EDGE_LOOP ( 'NONE', ( #83401, #83913 ) ) ;
#56567=CARTESIAN_POINT ( 'NONE',  ( 2.568367604407467919, -287.6537790870643789, -204.8731114234594202 ) ) ;
#56568=CARTESIAN_POINT ( 'NONE',  ( -79.07042575173363730, -279.8050455313261295, -210.4378258122584100 ) ) ;
#56569=CARTESIAN_POINT ( 'NONE',  ( -32.04762914715821864, -293.9072002357380029, -346.8822621854082513 ) ) ;
#56570=CARTESIAN_POINT ( 'NONE',  ( -44.40158332319210643, -283.7905138198533450, -346.9877081854161247 ) ) ;
#56571=CARTESIAN_POINT ( 'NONE',  ( -71.06079909490395607, -285.9525316224593894, -201.1602028402355984 ) ) ;
#56572=CARTESIAN_POINT ( 'NONE',  ( -48.32767700335139693, -283.5291232961614583, -342.5511158964246761 ) ) ;
#56573=CARTESIAN_POINT ( 'NONE',  ( 139.0626142690745723, 180.5554732948571655, -241.5151996274486237 ) ) ;
#56574=CARTESIAN_POINT ( 'NONE',  ( -110.7569340398763842, -265.4859700393970456, -306.5498943703896657 ) ) ;
#56575=CARTESIAN_POINT ( 'NONE',  ( 201.3568388210140370, 292.7455855533186195, -68.23575430854765500 ) ) ;
#56576=CARTESIAN_POINT ( 'NONE',  ( -2.828471751044380866, -273.7179372179217580, -205.8519031810168087 ) ) ;
#56577=CARTESIAN_POINT ( 'NONE',  ( 5.367948354894304330, -273.5654586165605906, -210.7155518452954936 ) ) ;
#56578=CARTESIAN_POINT ( 'NONE',  ( -92.65712151590203405, -295.3266424335277520, -323.8375713043415658 ) ) ;
#56579=CARTESIAN_POINT ( 'NONE',  ( -69.08132297861465076, -196.6430596737640712, -357.2208136483789076 ) ) ;
#56580=CARTESIAN_POINT ( 'NONE',  ( 19.67958836871779127, -273.5400615760668757, -219.2747051178490381 ) ) ;
#56581=CARTESIAN_POINT ( 'NONE',  ( -99.49450015584253038, -298.9668567094116725, -229.6737800469756792 ) ) ;
#56582=CARTESIAN_POINT ( 'NONE',  ( -62.92141544937182829, -292.7907688724012587, -201.6595587741367979 ) ) ;
#56584=CARTESIAN_POINT ( 'NONE',  ( -98.91092185458170150, -298.1052951054733740, -224.4910436230923949 ) ) ;
#56585=CARTESIAN_POINT ( 'NONE',  ( -10.69581716216383072, -289.1874996820229740, -338.4446794674656758 ) ) ;
#56586=CARTESIAN_POINT ( 'NONE',  ( 39.27927957544802240, -294.2825703586752866, -264.5832040531956295 ) ) ;
#56587=CARTESIAN_POINT ( 'NONE',  ( -96.46010517989168420, -296.3814511626835611, -319.6212304622717397 ) ) ;
#56588=CARTESIAN_POINT ( 'NONE',  ( 35.29510435112290168, -293.6164485697258897, -262.5998051288544843 ) ) ;
#56590=CARTESIAN_POINT ( 'NONE',  ( 37.94776876029222734, -277.5537237777252813, -276.7493940130202645 ) ) ;
#56592=CARTESIAN_POINT ( 'NONE',  ( -111.3830037309397341, -277.7974794228832707, -291.2755212521244061 ) ) ;
#56594=CARTESIAN_POINT ( 'NONE',  ( -8.890452257546689552, -275.3748145659170063, -202.8241881520525283 ) ) ;
#56595=CARTESIAN_POINT ( 'NONE',  ( -29.95992034420097383, -275.9045097189990656, -194.7338521300180787 ) ) ;
#56596=CARTESIAN_POINT ( 'NONE',  ( -111.6110347286899156, -276.7351536699262056, -257.6146383805146911 ) ) ;
#56597=CARTESIAN_POINT ( 'NONE',  ( -101.3077607516715943, -297.6865292886304815, -234.9741746814539169 ) ) ;
#56598=CARTESIAN_POINT ( 'NONE',  ( -82.73744520628724786, -294.2610853438101230, -328.3450185199600355 ) ) ;
#56600=CARTESIAN_POINT ( 'NONE',  ( -111.6732019855097917, -279.2939137386276798, -250.4518718852628467 ) ) ;
#56601=CARTESIAN_POINT ( 'NONE',  ( -40.50364157120243647, -277.2596628575806790, -343.3050716355485861 ) ) ;
#56603=CARTESIAN_POINT ( 'NONE',  ( 30.98891363689950751, -285.7913260709609062, -235.9485404281858223 ) ) ;
#56604=CARTESIAN_POINT ( 'NONE',  ( -36.93558507469707308, -300.0573805613046829, -195.1943045490916404 ) ) ;
#56606=CARTESIAN_POINT ( 'NONE',  ( 31.12933071685829134, -286.4044262406529811, -244.4436543141399625 ) ) ;
#56608=EDGE_CURVE ( 'NONE', #85445, #92893, #59148, .T. ) ;
#56609=CARTESIAN_POINT ( 'NONE',  ( 21.33280694625357654, -279.1655884264935139, -225.2264748078117123 ) ) ;
#56610=CARTESIAN_POINT ( 'NONE',  ( -109.4611051303957936, -277.3192106689721186, -255.6634924303688479 ) ) ;
#56611=CARTESIAN_POINT ( 'NONE',  ( -104.3187816133379897, -282.1993325540425417, -302.9662659308841626 ) ) ;
#56612=CARTESIAN_POINT ( 'NONE',  ( -84.69704586883723607, -287.4002016735916527, -212.1358925805832030 ) ) ;
#56613=CARTESIAN_POINT ( 'NONE',  ( 22.79997389512574557, -277.3418080879433205, -312.5210676675291666 ) ) ;
#56616=CARTESIAN_POINT ( 'NONE',  ( -105.4472355744958065, -276.3517999464380637, -304.1783846911034743 ) ) ;
#56617=CARTESIAN_POINT ( 'NONE',  ( 13.56169881221938489, -275.4397658221436131, -217.8945891822620808 ) ) ;
#56618=CARTESIAN_POINT ( 'NONE',  ( 29.08933421837456734, -283.0857735416603305, -235.0799766736670051 ) ) ;
#56620=CARTESIAN_POINT ( 'NONE',  ( 4.775329806740725935, -290.4082781498609620, -333.0944423448184466 ) ) ;
#56621=CARTESIAN_POINT ( 'NONE',  ( -104.9225891928995651, -294.9816826268902332, -237.7187071093943871 ) ) ;
#56622=AXIS2_PLACEMENT_3D ( 'NONE', #69668, #20428, #33210 ) ;
#56624=CARTESIAN_POINT ( 'NONE',  ( -38.07055923495801153, -272.7276544548315655, -196.8715796523499080 ) ) ;
#56625=CARTESIAN_POINT ( 'NONE',  ( 21.99514713599179672, -291.0757618644705644, -225.7516566589829381 ) ) ;
#56626=CARTESIAN_POINT ( 'NONE',  ( 172.7732574597264659, 233.5132621949535121, -195.2123807395911399 ) ) ;
#56628=CARTESIAN_POINT ( 'NONE',  ( -112.1917270975734624, -288.8439368079679070, -285.2659359728676236 ) ) ;
#56629=CARTESIAN_POINT ( 'NONE',  ( 36.73684395173320638, -285.5769064336103611, -253.3816119969115732 ) ) ;
#56631=CARTESIAN_POINT ( 'NONE',  ( -110.5827305937359881, -286.0775974361200724, -262.7066584158793603 ) ) ;
#56632=CARTESIAN_POINT ( 'NONE',  ( -90.85260795954805246, -284.6390734000214593, -320.2528454543183898 ) ) ;
#56633=CARTESIAN_POINT ( 'NONE',  ( -107.9418819357910451, -292.8741932966008221, -243.8680003984145799 ) ) ;
#56634=CARTESIAN_POINT ( 'NONE',  ( 26.42028899075831561, -274.1746367024695132, -311.0011806984875875 ) ) ;
#56635=CARTESIAN_POINT ( 'NONE',  ( 16.94332650267006457, -276.6379205362107427, -325.0146732586167104 ) ) ;
#56636=CARTESIAN_POINT ( 'NONE',  ( -104.7089585797346984, -289.0822963016607900, -236.0264345020260350 ) ) ;
#56637=CARTESIAN_POINT ( 'NONE',  ( -95.21079124202668709, -277.8647645372290071, -321.1564749913054015 ) ) ;
#56638=CARTESIAN_POINT ( 'NONE',  ( -66.67683049721047439, -297.4182497981705069, -339.0000058740760664 ) ) ;
#56641=CARTESIAN_POINT ( 'NONE',  ( -108.9093421591220192, -283.0173313112684923, -287.1289103747615741 ) ) ;
#56642=CARTESIAN_POINT ( 'NONE',  ( -98.60032658439844511, -277.1398641000526482, -227.0900960997149411 ) ) ;
#56644=CARTESIAN_POINT ( 'NONE',  ( 27.91971080898837698, -273.5100438833234762, -230.7169739896940257 ) ) ;
#56645=CARTESIAN_POINT ( 'NONE',  ( -96.17997698430839648, -277.2933346036577404, -313.7635487079500081 ) ) ;
#56646=CARTESIAN_POINT ( 'NONE',  ( 26.40199734520895802, -295.5748096586437441, -307.3401496571643179 ) ) ;
#56647=CARTESIAN_POINT ( 'NONE',  ( 3.668340451276424830, -279.5100976521551388, -205.4935287854272588 ) ) ;
#56648=CARTESIAN_POINT ( 'NONE',  ( -61.07813073046070684, -296.3091108082808773, -339.6968242111963150 ) ) ;
#56650=CARTESIAN_POINT ( 'NONE',  ( -92.33084088443780502, -297.1338721407038292, -323.5540937528919585 ) ) ;
#56651=CARTESIAN_POINT ( 'NONE',  ( -109.1497171808796338, -272.3972409699225636, -256.8356854507570119 ) ) ;
#56652=CARTESIAN_POINT ( 'NONE',  ( -67.38807564903632397, -293.6582444505723970, -201.6427363848794130 ) ) ;
#56653=CARTESIAN_POINT ( 'NONE',  ( -97.58172773319931537, -285.3609251400712310, -222.4013527759471174 ) ) ;
#56654=CARTESIAN_POINT ( 'NONE',  ( -36.92238861510700332, -272.1969721148030317, -194.5846314150446972 ) ) ;
#56655=CARTESIAN_POINT ( 'NONE',  ( 37.82448045515723578, -287.5951405168726183, -287.1259539487356847 ) ) ;
#56656=CARTESIAN_POINT ( 'NONE',  ( -97.75134497261254296, -281.1321173282420887, -226.5145489663710521 ) ) ;
#56657=CARTESIAN_POINT ( 'NONE',  ( -89.82313244521755280, -284.3478701727402154, -219.2089320493205378 ) ) ;
#56658=CARTESIAN_POINT ( 'NONE',  ( -96.59559146607324465, -287.9216386140500390, -316.3391237484386806 ) ) ;
#56659=CARTESIAN_POINT ( 'NONE',  ( -43.41528170534920861, -158.9639970630164498, -364.8434004397808508 ) ) ;
#56660=CARTESIAN_POINT ( 'NONE',  ( 18.71300612636314042, -286.3950498778984297, -223.4816383385648635 ) ) ;
#56661=CARTESIAN_POINT ( 'NONE',  ( -31.64176327053335669, -283.9231350776951217, -346.9271437445970037 ) ) ;
#56662=CARTESIAN_POINT ( 'NONE',  ( -112.0854227277996813, -289.8304251048978131, -252.8626567332632362 ) ) ;
#56663=CARTESIAN_POINT ( 'NONE',  ( -79.48547497314076793, -281.0937453553920022, -206.8128319637202992 ) ) ;
#56664=CARTESIAN_POINT ( 'NONE',  ( -113.2746445971862101, -279.7443217125004367, -280.1332313332333115 ) ) ;
#56665=CARTESIAN_POINT ( 'NONE',  ( 35.42883406461619700, -281.4697939825421713, -276.7532527611465412 ) ) ;
#56666=CARTESIAN_POINT ( 'NONE',  ( 34.00849916627620217, -277.8507559612054933, -293.4727970487795687 ) ) ;
#56667=CARTESIAN_POINT ( 'NONE',  ( -50.46752206666486273, -295.2151791643698857, -346.2880673641592466 ) ) ;
#56668=CARTESIAN_POINT ( 'NONE',  ( -97.90762704143034512, -287.9755737448996342, -313.9915580636235859 ) ) ;
#56669=CARTESIAN_POINT ( 'NONE',  ( -110.3568607010007980, -295.5658071095648438, -263.2560802976551599 ) ) ;
#56670=ORIENTED_EDGE ( 'NONE', *, *, #19214, .F. ) ;
#56672=CARTESIAN_POINT ( 'NONE',  ( 4.213975851907634684, -284.4078084029300726, -332.1846355355074820 ) ) ;
#56673=CARTESIAN_POINT ( 'NONE',  ( -86.50734310374677705, -295.4247318932015105, -324.3502561261821029 ) ) ;
#56674=CARTESIAN_POINT ( 'NONE',  ( 26.22893654932757457, -294.0632163582802718, -227.3693946471298659 ) ) ;
#56676=CARTESIAN_POINT ( 'NONE',  ( -8.446326822210314944, -283.3150140821632021, -337.5098340531724830 ) ) ;
#56677=CARTESIAN_POINT ( 'NONE',  ( -52.48743207520171694, -272.9216056904402876, -195.0511010066886968 ) ) ;
#56678=CARTESIAN_POINT ( 'NONE',  ( -91.52081670784414769, -290.4502124374193954, -325.0064848991340227 ) ) ;
#56679=CARTESIAN_POINT ( 'NONE',  ( -44.32927892556214999, -281.2790897366164700, -345.8555132341144258 ) ) ;
#56680=CARTESIAN_POINT ( 'NONE',  ( -114.3477987538904870, -290.9104725861690781, -268.3594982842531067 ) ) ;
#56681=CARTESIAN_POINT ( 'NONE',  ( -18.46394633714706757, -289.1355902506487041, -340.9524886010027558 ) ) ;
#56683=FACE_OUTER_BOUND ( 'NONE', #55277, .T. ) ;
#56684=CARTESIAN_POINT ( 'NONE',  ( 189.0190693845576391, 268.0883035360336635, -137.5188113462812680 ) ) ;
#56685=CARTESIAN_POINT ( 'NONE',  ( -95.95921662488163406, -288.6952119285919025, -223.5744983911110353 ) ) ;
#56687=CARTESIAN_POINT ( 'NONE',  ( -96.64771065340420364, -278.0730481389181250, -227.2679260633267404 ) ) ;
#56688=CARTESIAN_POINT ( 'NONE',  ( 4.855119491839677615, -274.2717736081243061, -205.9148560242031465 ) ) ;
#56689=CARTESIAN_POINT ( 'NONE',  ( -111.9953344657296270, -280.4765637467240822, -276.2478437392741739 ) ) ;
#56690=CARTESIAN_POINT ( 'NONE',  ( -106.9267777310214598, -266.4941316993138685, -306.1134506589970101 ) ) ;
#56691=CARTESIAN_POINT ( 'NONE',  ( 25.80400527064101723, -279.5540061349556140, -227.2428875975125209 ) ) ;
#56692=CARTESIAN_POINT ( 'NONE',  ( -37.57032110175317285, -281.0751734034562901, -345.0182820352854378 ) ) ;
#56693=CARTESIAN_POINT ( 'NONE',  ( -105.6128327790994206, -298.7463959362008836, -236.9990668191579744 ) ) ;
#56695=CARTESIAN_POINT ( 'NONE',  ( 35.68263806977347485, -294.0137760869725980, -268.0299225310544671 ) ) ;
#56697=CARTESIAN_POINT ( 'NONE',  ( -108.5824064054046119, -289.4742857532162930, -252.2543676344083394 ) ) ;
#56698=CARTESIAN_POINT ( 'NONE',  ( 4.800355109748853266, -275.2563093750758867, -205.9756310118413580 ) ) ;
#56699=CARTESIAN_POINT ( 'NONE',  ( -68.28257698571616174, -273.6341103214037958, -204.2288740640422304 ) ) ;
#56704=CARTESIAN_POINT ( 'NONE',  ( -41.08064305408498740, -281.0836649227019848, -197.1474144842652834 ) ) ;
#56705=CARTESIAN_POINT ( 'NONE',  ( -97.78413017831341847, -280.9345627693524534, -224.2890008721304014 ) ) ;
#56706=CARTESIAN_POINT ( 'NONE',  ( -106.3996038924070149, -283.2856876924329299, -294.8928170414952774 ) ) ;
#56707=CARTESIAN_POINT ( 'NONE',  ( 35.77974035929660346, -283.2463849577728183, -257.5501686496451157 ) ) ;
#56708=CARTESIAN_POINT ( 'NONE',  ( 33.53213756393575551, -273.7654484043518437, -249.9893292490428678 ) ) ;
#56711=CARTESIAN_POINT ( 'NONE',  ( -101.9556507943157584, -278.8071245518754608, -312.0417934033824281 ) ) ;
#56715=CARTESIAN_POINT ( 'NONE',  ( -49.79628808495661474, -285.1900151265476211, -344.7326805636440099 ) ) ;
#56716=CARTESIAN_POINT ( 'NONE',  ( 21.12900100429709127, -292.1331741950734795, -226.3863657205809830 ) ) ;
#56717=CARTESIAN_POINT ( 'NONE',  ( -12.26481900721097951, -288.0830187269731937, -343.1112238485928856 ) ) ;
#56719=CARTESIAN_POINT ( 'NONE',  ( -97.38393068692143117, -283.3891947413420098, -227.0624381932072140 ) ) ;
#56720=CARTESIAN_POINT ( 'NONE',  ( -97.04230389957892555, -283.7240095705122940, -227.3139050342514622 ) ) ;
#56721=CARTESIAN_POINT ( 'NONE',  ( -81.02338749182996480, -287.8939974727422850, -330.1734152387459176 ) ) ;
#56722=CARTESIAN_POINT ( 'NONE',  ( -26.66995869052062673, -284.1186018979579444, -343.0298064703055161 ) ) ;
#56723=CARTESIAN_POINT ( 'NONE',  ( -16.31305462463360101, -272.3236647156698496, -198.3155668041703166 ) ) ;
#56724=CARTESIAN_POINT ( 'NONE',  ( -113.0226960804680800, -283.0642294492725455, -261.4826459136350536 ) ) ;
#56725=CARTESIAN_POINT ( 'NONE',  ( -107.5559382861217159, -298.2082499079031663, -296.8696270065109957 ) ) ;
#56726=CARTESIAN_POINT ( 'NONE',  ( -107.3123243349159566, -282.9102301238597761, -242.7580784090494603 ) ) ;
#56727=CARTESIAN_POINT ( 'NONE',  ( -107.4558385693462981, -279.7725523539320420, -249.2089067747869251 ) ) ;
#56728=CARTESIAN_POINT ( 'NONE',  ( 18.89770494555045488, -288.8595077096412638, -220.4129036198637550 ) ) ;
#56731=CARTESIAN_POINT ( 'NONE',  ( 14.50864081789039162, -296.2495432193971965, -325.3234354361447913 ) ) ;
#56732=CARTESIAN_POINT ( 'NONE',  ( -42.00572826972197049, -275.1107534575936029, -345.2289022584454301 ) ) ;
#56733=CARTESIAN_POINT ( 'NONE',  ( -114.2286627002245893, -289.7385977494367921, -271.2167335908632140 ) ) ;
#56734=CARTESIAN_POINT ( 'NONE',  ( 20.30603714499941859, -292.5960922907211739, -316.4592202991721024 ) ) ;
#56735=CARTESIAN_POINT ( 'NONE',  ( -27.47570216592813352, -278.8647953589371582, -197.4816625090732884 ) ) ;
#56736=CARTESIAN_POINT ( 'NONE',  ( -75.83114612811395716, -295.6724034417384814, -206.8237537036981166 ) ) ;
#56737=CARTESIAN_POINT ( 'NONE',  ( -55.14793967977271905, -293.1334808871755513, -199.0576726967778711 ) ) ;
#56738=CARTESIAN_POINT ( 'NONE',  ( 31.98288692825981272, -284.4805209788416391, -303.7098442033570223 ) ) ;
#56739=CARTESIAN_POINT ( 'NONE',  ( -112.9123887431978233, -295.1666498957275167, -259.6942202617385647 ) ) ;
#56740=CARTESIAN_POINT ( 'NONE',  ( 21.82696275339847602, -289.7646664163939931, -314.4902125429033504 ) ) ;
#56741=CARTESIAN_POINT ( 'NONE',  ( -50.37028049401970975, -290.1278643719413708, -195.4997120031707993 ) ) ;
#56744=CARTESIAN_POINT ( 'NONE',  ( -109.0054099783330486, -292.1969947538240149, -253.5822444988266113 ) ) ;
#56747=CARTESIAN_POINT ( 'NONE',  ( -91.80017830655891942, -292.0528026991282218, -221.4867128888363368 ) ) ;
#56748=CARTESIAN_POINT ( 'NONE',  ( 128.9960186029002500, -299.5541904835127980, -195.3611179825600175 ) ) ;
#56749=CARTESIAN_POINT ( 'NONE',  ( -112.5381414619063207, -291.9417703719585688, -255.6809424883213069 ) ) ;
#56750=CARTESIAN_POINT ( 'NONE',  ( 30.55075662629251099, -279.1422954241611478, -237.5450997411538765 ) ) ;
#56751=CARTESIAN_POINT ( 'NONE',  ( 31.80103605861241078, -293.2391603830303666, -246.7883386583480387 ) ) ;
#56752=CARTESIAN_POINT ( 'NONE',  ( 39.71044205758624912, -281.5467637937352947, -269.9302679464767039 ) ) ;
#56753=CARTESIAN_POINT ( 'NONE',  ( 34.56624224448843563, -281.5668343145136419, -297.8382378316797485 ) ) ;
#56755=CARTESIAN_POINT ( 'NONE',  ( 26.67062851513158250, -285.0279146717099934, -231.2788658862751561 ) ) ;
#56756=CARTESIAN_POINT ( 'NONE',  ( 34.51323068508828129, -279.9344127122364512, -289.0593257110613763 ) ) ;
#56757=CARTESIAN_POINT ( 'NONE',  ( -107.1571581817064782, -282.9102301224093026, -242.8192301167730420 ) ) ;
#56758=LINE ( 'NONE', #20285, #74461 ) ;
#56759=CARTESIAN_POINT ( 'NONE',  ( -25.48406923646075484, -278.6805263413885427, -194.9813836975748416 ) ) ;
#56761=CARTESIAN_POINT ( 'NONE',  ( 14.04997972262696670, -285.6736460602409124, -213.3654549563043474 ) ) ;
#56762=CARTESIAN_POINT ( 'NONE',  ( -19.24153929570557509, -275.0937682714692301, -199.4214417295161184 ) ) ;
#56764=CARTESIAN_POINT ( 'NONE',  ( 36.42027776062617761, -295.1213789819406657, -267.9923564776565854 ) ) ;
#56765=CARTESIAN_POINT ( 'NONE',  ( -10.57118739194255674, -275.8197702734472045, -198.7370626128347055 ) ) ;
#56766=CARTESIAN_POINT ( 'NONE',  ( -39.16254299575933828, -276.7423474558363523, -343.3595564460371179 ) ) ;
#56767=CARTESIAN_POINT ( 'NONE',  ( -107.2613205284957729, -291.1328495609135985, -237.9812195377652699 ) ) ;
#56768=CARTESIAN_POINT ( 'NONE',  ( 36.72900442108796426, -279.8222554896709653, -285.2891094308296260 ) ) ;
#56769=CARTESIAN_POINT ( 'NONE',  ( 29.47669420865653933, -292.8883005951869904, -232.0949164105482794 ) ) ;
#56770=CARTESIAN_POINT ( 'NONE',  ( -52.40650087544421609, -290.9133393305313575, -198.6399494117271445 ) ) ;
#56771=CARTESIAN_POINT ( 'NONE',  ( 31.56862506508735677, -291.9406376160899299, -300.0956789718887876 ) ) ;
#56774=CARTESIAN_POINT ( 'NONE',  ( 29.91484724564734066, -292.6753985979214008, -241.6914185068661709 ) ) ;
#56776=CARTESIAN_POINT ( 'NONE',  ( -92.05005921254146983, -276.6952119285918457, -226.6919474004047572 ) ) ;
#56777=CARTESIAN_POINT ( 'NONE',  ( -109.6252612907722579, -295.9381362787688090, -244.5172212517033756 ) ) ;
#56778=CARTESIAN_POINT ( 'NONE',  ( -103.6216568320890445, -286.3684757066138218, -232.0423045623604992 ) ) ;
#56779=CARTESIAN_POINT ( 'NONE',  ( 17.77758282519474520, -286.7031433577826078, -222.4981401057240760 ) ) ;
#56780=CARTESIAN_POINT ( 'NONE',  ( -24.18700188309069787, -278.4014013403927947, -342.9227942856481945 ) ) ;
#56781=CARTESIAN_POINT ( 'NONE',  ( -111.4403711765601344, -294.4506259081986173, -279.7891289446308178 ) ) ;
#56782=CARTESIAN_POINT ( 'NONE',  ( -110.8075262018316351, -298.1900563010285623, -279.7564097233081952 ) ) ;
#56783=CARTESIAN_POINT ( 'NONE',  ( 35.09652309596444297, -274.5062457632989776, -282.4929824959415896 ) ) ;
#56786=CARTESIAN_POINT ( 'NONE',  ( -77.07495303850760138, -295.2356076050358524, -336.3550143346614618 ) ) ;
#56787=CARTESIAN_POINT ( 'NONE',  ( 30.75200374132935721, -289.8707168858433079, -300.5650338641434587 ) ) ;
#56788=CARTESIAN_POINT ( 'NONE',  ( 202.9738562182569694, 295.9636489450776367, -54.00000000004089173 ) ) ;
#56789=CARTESIAN_POINT ( 'NONE',  ( -63.85013099144709514, -290.0584419598487784, -338.5416980120431845 ) ) ;
#56791=CARTESIAN_POINT ( 'NONE',  ( -8.936999191915294460, -279.4735078222589095, -199.0449684947067226 ) ) ;
#56792=CARTESIAN_POINT ( 'NONE',  ( -103.7659439306353306, -297.7095486230705887, -231.5117085965722765 ) ) ;
#56793=CARTESIAN_POINT ( 'NONE',  ( -111.7079305856647551, -288.8767743187848964, -255.8033243646799519 ) ) ;
#56794=CARTESIAN_POINT ( 'NONE',  ( -98.25512482786351143, -296.2569967246311080, -317.4280807376011921 ) ) ;
#56795=CARTESIAN_POINT ( 'NONE',  ( 12.37237532559006148, -294.6703387249092430, -323.9149846298220154 ) ) ;
#56798=CARTESIAN_POINT ( 'NONE',  ( 36.47863337052626775, -289.3163021980049052, -289.6812141656515109 ) ) ;
#56799=CARTESIAN_POINT ( 'NONE',  ( -37.30987171927208834, -295.5523547857347353, -190.3611179825600175 ) ) ;
#56801=CARTESIAN_POINT ( 'NONE',  ( 36.08085304393108572, -280.6132212610799002, -247.5041393481000398 ) ) ;
#56802=CARTESIAN_POINT ( 'NONE',  ( -100.5666733072493173, -286.0114868529720411, -310.4909528210415033 ) ) ;
#56803=CARTESIAN_POINT ( 'NONE',  ( -15.56388324074766594, -284.9031953737429035, -197.0645381205981437 ) ) ;
#56804=CARTESIAN_POINT ( 'NONE',  ( -75.47415218002545600, -287.6447520726788980, -334.3075471078943224 ) ) ;
#56805=CARTESIAN_POINT ( 'NONE',  ( 32.56456143457394603, -277.0334261622098211, -241.0123647036332102 ) ) ;
#56807=CARTESIAN_POINT ( 'NONE',  ( -109.2860834537281107, -278.3880026119782656, -282.8045513793434225 ) ) ;
#56808=CARTESIAN_POINT ( 'NONE',  ( 34.58425318030838014, -281.0736959019765777, -283.4906920588849175 ) ) ;
#56809=CARTESIAN_POINT ( 'NONE',  ( 34.42762214996863435, -276.2884572016843094, -243.3304522691763054 ) ) ;
#56810=CARTESIAN_POINT ( 'NONE',  ( -111.6967694131591742, -277.5793378866123362, -251.8863690268112805 ) ) ;
#56811=CARTESIAN_POINT ( 'NONE',  ( 201.0615148111058375, 294.6280088066692997, -54.00000000000862599 ) ) ;
#56812=CARTESIAN_POINT ( 'NONE',  ( -113.9471166701324023, -273.5649751209182909, -264.6557064416240337 ) ) ;
#56814=CARTESIAN_POINT ( 'NONE',  ( 7.540083511923226567, -300.0289523866539412, -193.9397036489160087 ) ) ;
#56815=CARTESIAN_POINT ( 'NONE',  ( -54.42813229853333468, -285.7662352645560873, -345.3683826091709648 ) ) ;
#56817=CARTESIAN_POINT ( 'NONE',  ( 82.62398566199905758, -301.5110966808080093, -193.7954372207628069 ) ) ;
#56818=CARTESIAN_POINT ( 'NONE',  ( 27.30953247925155836, -289.1022317698025290, -305.0299284288985291 ) ) ;
#56819=CARTESIAN_POINT ( 'NONE',  ( -29.58890784089300752, -287.9091986229846611, -194.7709848651294919 ) ) ;
#56820=CARTESIAN_POINT ( 'NONE',  ( 34.09738485971947597, -286.6965092121349699, -254.8578988116283597 ) ) ;
#56821=CARTESIAN_POINT ( 'NONE',  ( -12.79777069895160935, -294.3712007776510973, -199.4370578810420795 ) ) ;
#56822=CARTESIAN_POINT ( 'NONE',  ( -93.39100730602349643, -283.3396800105341526, -323.0871895847829478 ) ) ;
#56823=CARTESIAN_POINT ( 'NONE',  ( -7.659186173002896503, -278.8476830580592036, -202.7796329416476055 ) ) ;
#56824=CARTESIAN_POINT ( 'NONE',  ( -19.54225204922731152, -288.1439343479934792, -198.2913939261817404 ) ) ;
#56825=CARTESIAN_POINT ( 'NONE',  ( 28.40866685983767326, -279.5830819510757692, -236.9673319692633129 ) ) ;
#56826=CARTESIAN_POINT ( 'NONE',  ( -41.87035152653127312, -278.4255526404249963, -343.7272915648097182 ) ) ;
#56827=CARTESIAN_POINT ( 'NONE',  ( -8.952702767496232283, -274.9259822828680626, -202.9866371157663707 ) ) ;
#56828=CARTESIAN_POINT ( 'NONE',  ( -26.21745756478734179, -287.7084680293881433, -346.1520141715661225 ) ) ;
#56830=CARTESIAN_POINT ( 'NONE',  ( -83.77746811494833423, -284.4739443136207910, -331.6478663621231817 ) ) ;
#56831=CARTESIAN_POINT ( 'NONE',  ( -71.70562383742948498, -283.9864296807396045, -339.1989538783423654 ) ) ;
#56832=CARTESIAN_POINT ( 'NONE',  ( 34.23110049439648606, -281.9091522222768731, -284.7883723717259841 ) ) ;
#56835=FACE_OUTER_BOUND ( 'NONE', #25685, .T. ) ;
#56836=CARTESIAN_POINT ( 'NONE',  ( 2.550249945180924627, -290.3842292782780419, -334.8349224950468397 ) ) ;
#56837=CARTESIAN_POINT ( 'NONE',  ( -1.023102048212159998, -291.2087973157287593, -203.0242209119136305 ) ) ;
#56838=CARTESIAN_POINT ( 'NONE',  ( -74.38207326934181651, -272.6056845373276474, -207.1246984394913682 ) ) ;
#56839=CARTESIAN_POINT ( 'NONE',  ( 21.28455134861987474, -293.5724245778756654, -320.1233066875379336 ) ) ;
#56840=CARTESIAN_POINT ( 'NONE',  ( -109.8646543130901279, -288.8610817458686029, -283.4427413478246081 ) ) ;
#56841=CARTESIAN_POINT ( 'NONE',  ( 21.31273283856296885, -292.4188606709935812, -315.5219929201330729 ) ) ;
#56842=CARTESIAN_POINT ( 'NONE',  ( 36.07712869506050879, -288.7300087896967966, -268.2860053273743688 ) ) ;
#56843=CARTESIAN_POINT ( 'NONE',  ( 10.64812456238590066, -290.9090924074130839, -330.4860931364851808 ) ) ;
#56844=CARTESIAN_POINT ( 'NONE',  ( -68.50249632939708988, -291.4617104047676435, -338.5954357219931694 ) ) ;
#56845=CARTESIAN_POINT ( 'NONE',  ( -101.6342081159107948, -289.0738365943886947, -231.3185312610129927 ) ) ;
#56846=CARTESIAN_POINT ( 'NONE',  ( -53.73033226344534086, -293.8421367365797323, -197.1210015038540178 ) ) ;
#56847=CARTESIAN_POINT ( 'NONE',  ( -72.49746091384216129, -286.5159606300380233, -206.1013805704130846 ) ) ;
#56848=CARTESIAN_POINT ( 'NONE',  ( 36.51891599923905574, -295.3735751992887799, -256.4098522915998046 ) ) ;
#56849=CARTESIAN_POINT ( 'NONE',  ( -113.6885439307725818, -271.0584006130368380, -270.3420989471088660 ) ) ;
#56851=CARTESIAN_POINT ( 'NONE',  ( -70.69790813302894605, -275.5942986426687185, -202.7906348204811877 ) ) ;
#56852=CARTESIAN_POINT ( 'NONE',  ( -15.57575551524399238, -280.7703005209700677, -342.1332873906470127 ) ) ;
#56853=CARTESIAN_POINT ( 'NONE',  ( -111.8146800288023286, -295.5114887909660979, -289.3334102642808716 ) ) ;
#56854=CARTESIAN_POINT ( 'NONE',  ( -49.01343685127250893, -272.1414185873658198, -197.2219963520723525 ) ) ;
#56855=CARTESIAN_POINT ( 'NONE',  ( -106.8502854795440413, -276.9826370022785227, -243.5734670331097504 ) ) ;
#56856=CARTESIAN_POINT ( 'NONE',  ( -51.65383020848835827, -275.0702021452863164, -198.3208966084563656 ) ) ;
#56857=CARTESIAN_POINT ( 'NONE',  ( 25.66903081692104038, -273.5518117621004421, -227.1146142734469038 ) ) ;
#56858=CARTESIAN_POINT ( 'NONE',  ( -96.06363718400488949, -297.3591076226111909, -314.7339728661498839 ) ) ;
#56860=CARTESIAN_POINT ( 'NONE',  ( -108.7472414845238973, -297.1452719126152715, -286.2938010946481882 ) ) ;
#56861=CARTESIAN_POINT ( 'NONE',  ( -112.3417001280820386, -272.5521521680024648, -270.3611179825637691 ) ) ;
#56862=CARTESIAN_POINT ( 'NONE',  ( 22.56941999757815864, -284.9493879587978995, -224.6336679413746538 ) ) ;
#56863=CARTESIAN_POINT ( 'NONE',  ( -109.5824463581982542, -272.5285553788712036, -259.5145635099089532 ) ) ;
#56864=CARTESIAN_POINT ( 'NONE',  ( -20.98396659394967045, -286.2564902239945468, -195.1186794679401828 ) ) ;
#56865=CARTESIAN_POINT ( 'NONE',  ( 20.55419534580220287, -287.9056177152211831, -321.1137015996543482 ) ) ;
#56866=CARTESIAN_POINT ( 'NONE',  ( -90.49361667431075773, -299.2837399151713385, -216.9450102151081410 ) ) ;
#56867=CARTESIAN_POINT ( 'NONE',  ( 19.34493790852515360, -292.2309370920916081, -319.2340354594890073 ) ) ;
#56868=CARTESIAN_POINT ( 'NONE',  ( -68.59745950965171346, -278.8489373814357464, -200.1524878548045763 ) ) ;
#56869=CARTESIAN_POINT ( 'NONE',  ( -54.42813229853332757, -289.3380690714490129, -195.3538533559490702 ) ) ;
#56871=CARTESIAN_POINT ( 'NONE',  ( 8.214463808611272455, -287.2076671594689969, -327.9090669553941666 ) ) ;
#56874=CARTESIAN_POINT ( 'NONE',  ( -15.28719573718626457, -286.7665914097424888, -342.0994090541371406 ) ) ;
#56875=CARTESIAN_POINT ( 'NONE',  ( -94.32674145552130085, -274.7281231926065743, -223.6143778571423013 ) ) ;
#56876=CARTESIAN_POINT ( 'NONE',  ( 8.180831956586883891, -282.0860793272931915, -208.9251251742019235 ) ) ;
#56877=CARTESIAN_POINT ( 'NONE',  ( -78.59798690511595964, -293.6248854651838656, -333.4192308821029087 ) ) ;
#56878=CARTESIAN_POINT ( 'NONE',  ( 22.58477221173992078, -282.1331888100040146, -312.0482612392601709 ) ) ;
#56879=CARTESIAN_POINT ( 'NONE',  ( -99.92278962374336970, -297.3133179158986081, -225.4990266129764507 ) ) ;
#56880=CARTESIAN_POINT ( 'NONE',  ( -99.79002154730132190, -274.5104264878792719, -231.4306406096073658 ) ) ;
#56882=CARTESIAN_POINT ( 'NONE',  ( 36.81324051993287583, -283.4038447052250262, -258.7980346704216572 ) ) ;
#56883=CARTESIAN_POINT ( 'NONE',  ( -109.0069000545257438, -295.8100095338479605, -255.2175149702159445 ) ) ;
#56886=CARTESIAN_POINT ( 'NONE',  ( 21.49261924077924135, -284.1652513568672589, -316.2998779917808747 ) ) ;
#56887=DIRECTION ( 'NONE',  ( 0.9951408606192334583, 1.205805641958521361E-17, 0.09846150276129006507 ) ) ;
#56888=CARTESIAN_POINT ( 'NONE',  ( 31.95455697924147032, -285.4809262143061801, -303.7686719486574702 ) ) ;
#56889=CARTESIAN_POINT ( 'NONE',  ( -1.552024450238887354, -275.7870919687083529, -338.3556614091436359 ) ) ;
#56890=CARTESIAN_POINT ( 'NONE',  ( 6.677930937926969790, -292.5033594675655308, -212.1264883770056713 ) ) ;
#56891=CARTESIAN_POINT ( 'NONE',  ( 21.05357421902077419, -282.4453198092525668, -225.3884229207988312 ) ) ;
#56893=CARTESIAN_POINT ( 'NONE',  ( 35.50010056705049521, -277.3109969259734839, -282.5242107043105761 ) ) ;
#56894=CARTESIAN_POINT ( 'NONE',  ( -111.9458314826517409, -285.7692499673535735, -286.8786807654246331 ) ) ;
#56895=CARTESIAN_POINT ( 'NONE',  ( 34.87338347557749074, -280.5201228497765555, -283.5506168502577111 ) ) ;
#56896=CARTESIAN_POINT ( 'NONE',  ( -96.84463670779649647, -279.9270754050482992, -316.0163607360962601 ) ) ;
#56897=CARTESIAN_POINT ( 'NONE',  ( -37.25358771661635160, -298.0532286319332798, -193.3603543084721821 ) ) ;
#56898=CARTESIAN_POINT ( 'NONE',  ( 38.18195486687699258, -275.5731426814587621, -285.3670348398762258 ) ) ;
#56899=CARTESIAN_POINT ( 'NONE',  ( 29.70191190629370581, -295.9030012171571116, -302.8292357805218558 ) ) ;
#56902=CARTESIAN_POINT ( 'NONE',  ( -107.2447219181401294, -294.3124804704074791, -299.7181098438056210 ) ) ;
#56903=CARTESIAN_POINT ( 'NONE',  ( 30.23412476943069649, -274.6862616529999741, -242.4524217175309957 ) ) ;
#56904=CARTESIAN_POINT ( 'NONE',  ( 37.11174518959666813, -295.2839562669528277, -287.1351906181812410 ) ) ;
#56905=CARTESIAN_POINT ( 'NONE',  ( 35.11586680115529902, -295.0739691744238371, -295.3815541510010121 ) ) ;
#56906=CARTESIAN_POINT ( 'NONE',  ( 34.07063134419961870, -289.8434941292947542, -292.9013247801119064 ) ) ;
#56907=CARTESIAN_POINT ( 'NONE',  ( -51.65590036480032410, -275.2355271501059519, -343.8126809006914755 ) ) ;
#56908=CARTESIAN_POINT ( 'NONE',  ( 1.646058413034991785, -278.4470922088816565, -333.8351728074196103 ) ) ;
#56909=CARTESIAN_POINT ( 'NONE',  ( -37.01327804955438694, -293.1278232743370040, -344.8130663223228680 ) ) ;
#56910=CARTESIAN_POINT ( 'NONE',  ( 32.43771646870996506, -283.7958510998655015, -300.0102549838469486 ) ) ;
#56911=CARTESIAN_POINT ( 'NONE',  ( -102.5069106769047096, -283.9270790817337229, -236.7795544871026721 ) ) ;
#56912=CARTESIAN_POINT ( 'NONE',  ( 123.5159050921753732, 147.8964653910322227, -262.5416932347842476 ) ) ;
#56913=CARTESIAN_POINT ( 'NONE',  ( -69.98807517729166250, -285.2765890292004087, -205.0302375404852171 ) ) ;
#56915=CARTESIAN_POINT ( 'NONE',  ( 27.58231245809937704, -282.0940213766514262, -229.4404881202036393 ) ) ;
#56916=CARTESIAN_POINT ( 'NONE',  ( -112.1407119049886489, -283.1393277365581298, -286.8873564434757100 ) ) ;
#56917=CARTESIAN_POINT ( 'NONE',  ( -92.91172984244634847, -280.2203447056240293, -217.3248688841182457 ) ) ;
#56918=( NAMED_UNIT ( * ) PLANE_ANGLE_UNIT ( ) SI_UNIT ( $, .RADIAN. ) );
#56919=CARTESIAN_POINT ( 'NONE',  ( -104.3573546980911573, -279.5957396292412227, -306.8523469782555821 ) ) ;
#56920=CARTESIAN_POINT ( 'NONE',  ( -92.08974858914540107, -275.4094976428775681, -313.9805196606274080 ) ) ;
#56921=CARTESIAN_POINT ( 'NONE',  ( -111.8162934558724686, -271.8246563314528430, -296.4050190923600212 ) ) ;
#56923=CARTESIAN_POINT ( 'NONE',  ( 54.71294253227434012, -301.2046906602610647, -195.3297278719368251 ) ) ;
#56924=CARTESIAN_POINT ( 'NONE',  ( 197.0526034356285834, 285.3763918474514867, -111.7597976793902745 ) ) ;
#56925=CARTESIAN_POINT ( 'NONE',  ( -21.82849779101435672, -278.2718982304160704, -197.2931086138896433 ) ) ;
#56926=CARTESIAN_POINT ( 'NONE',  ( -100.8495406482632006, -292.8691193047577030, -228.5446216049518000 ) ) ;
#56927=CARTESIAN_POINT ( 'NONE',  ( 23.43059176747042116, -292.3373188057852872, -229.7332801619119493 ) ) ;
#56928=CARTESIAN_POINT ( 'NONE',  ( -43.18388136776747643, -288.6317150851102156, -347.0774514559837485 ) ) ;
#56931=CARTESIAN_POINT ( 'NONE',  ( 20.90661756809265626, -292.7986906188394300, -319.8155392203443625 ) ) ;
#56932=CARTESIAN_POINT ( 'NONE',  ( -37.25974681457593363, -284.4530287867748370, -196.5485861912586927 ) ) ;
#56933=CARTESIAN_POINT ( 'NONE',  ( -86.76881564727500518, -293.2169640281572924, -214.9039522005589333 ) ) ;
#56934=CARTESIAN_POINT ( 'NONE',  ( 32.70642831699704800, -283.1621450715470019, -292.7644115030059879 ) ) ;
#56936=CARTESIAN_POINT ( 'NONE',  ( -112.0909025917204787, -291.7126243299221073, -252.8860802084473391 ) ) ;
#56937=CARTESIAN_POINT ( 'NONE',  ( -1.941747386683363219, -281.0269234322302623, -206.4484291980828345 ) ) ;
#56938=CARTESIAN_POINT ( 'NONE',  ( 34.07573131882021755, -292.6999002978242288, -298.0659768212267977 ) ) ;
#56939=CARTESIAN_POINT ( 'NONE',  ( 37.34987216221739459, -288.5816919551905926, -288.4535802332993626 ) ) ;
#56940=CARTESIAN_POINT ( 'NONE',  ( -70.60678316172038649, -289.9713676323442542, -339.7511000828700958 ) ) ;
#56941=CARTESIAN_POINT ( 'NONE',  ( 31.40011387464588211, -288.0459424448731056, -294.9286374363081791 ) ) ;
#56944=CARTESIAN_POINT ( 'NONE',  ( -11.45658210774083230, -296.5790722088510165, -341.6225882980729693 ) ) ;
#56945=CARTESIAN_POINT ( 'NONE',  ( -91.27593461744098136, -295.9892048044292778, -216.0988233189382868 ) ) ;
#56946=CARTESIAN_POINT ( 'NONE',  ( -87.26465425291733879, -276.8276912394720171, -323.9438306713270208 ) ) ;
#56947=CARTESIAN_POINT ( 'NONE',  ( -99.51361648575650065, -272.6628428023130937, -224.9497257201346940 ) ) ;
#56948=CARTESIAN_POINT ( 'NONE',  ( -93.62433890005128490, -294.3621618978256151, -317.9513820634163039 ) ) ;
#56949=CARTESIAN_POINT ( 'NONE',  ( 20.83266759778180699, -277.9490847756807739, -316.1386876423610488 ) ) ;
#56950=CARTESIAN_POINT ( 'NONE',  ( -50.10696186630607940, -296.1268671890846917, -197.4569198592163275 ) ) ;
#56951=CARTESIAN_POINT ( 'NONE',  ( 35.82146021440599526, -294.8340551310141677, -276.2162416171337895 ) ) ;
#56952=CARTESIAN_POINT ( 'NONE',  ( -94.17349107486099058, -296.9788784132343267, -316.6882248832757227 ) ) ;
#56954=CARTESIAN_POINT ( 'NONE',  ( -112.5044686842429371, -294.5618006923252210, -269.5951895088238643 ) ) ;
#56955=CARTESIAN_POINT ( 'NONE',  ( -36.55026780097767869, -298.7132266003461609, -193.4629651673951400 ) ) ;
#56956=CARTESIAN_POINT ( 'NONE',  ( -64.05155414336680053, -287.9820915129198511, -338.9865755659113233 ) ) ;
#56957=CARTESIAN_POINT ( 'NONE',  ( -77.66027734927040171, -275.5109923772375851, -207.1202057633774416 ) ) ;
#56958=CARTESIAN_POINT ( 'NONE',  ( -68.82462314344466847, -274.1416028730830590, -200.1445082283984505 ) ) ;
#56959=CARTESIAN_POINT ( 'NONE',  ( -95.30844261486753055, -297.5101944152214628, -225.9341639076047272 ) ) ;
#56960=CARTESIAN_POINT ( 'NONE',  ( -70.53332434206403434, -281.5965882558043063, -202.7096369237689828 ) ) ;
#56961=CARTESIAN_POINT ( 'NONE',  ( 31.93866299124532304, -280.6566962819538276, -302.9439941192916308 ) ) ;
#56962=EDGE_LOOP ( 'NONE', ( #70327, #35935, #42418, #4009 ) ) ;
#56963=CARTESIAN_POINT ( 'NONE',  ( 6.859627982674678215, -281.8169376483469364, -333.3512253923741468 ) ) ;
#56964=CARTESIAN_POINT ( 'NONE',  ( 33.62268972732272942, -274.5220013279320028, -240.6031520531212777 ) ) ;
#56965=CARTESIAN_POINT ( 'NONE',  ( -1.493590280205330689, -278.9192612726224070, -203.1201078980975581 ) ) ;
#56966=CARTESIAN_POINT ( 'NONE',  ( -96.24399245295794003, -277.1921505458130923, -223.6647756166170495 ) ) ;
#56967=CARTESIAN_POINT ( 'NONE',  ( -5.033110370024855840, -273.0607859142414782, -204.2296337750664748 ) ) ;
#56968=CARTESIAN_POINT ( 'NONE',  ( -37.67496901067786297, -276.0481711635446800, -195.3492686136225700 ) ) ;
#56971=CARTESIAN_POINT ( 'NONE',  ( 34.72157659004641772, -291.2896214802218537, -248.3317977032069450 ) ) ;
#56972=CARTESIAN_POINT ( 'NONE',  ( -30.69726913359199116, -292.1338189861018009, -193.5955736811883128 ) ) ;
#56973=CARTESIAN_POINT ( 'NONE',  ( -17.80916112088869951, -278.8009893514287114, -342.9456090505674410 ) ) ;
#56974=CARTESIAN_POINT ( 'NONE',  ( -0.7245070546902723230, -272.5383256351898922, -204.8927484250020541 ) ) ;
#56977=CARTESIAN_POINT ( 'NONE',  ( -70.69899523382866846, -283.6121493955225219, -203.1734501447768650 ) ) ;
#56979=CARTESIAN_POINT ( 'NONE',  ( 10.53901234483598337, -293.1681233877403088, -325.9899583156043832 ) ) ;
#56980=CARTESIAN_POINT ( 'NONE',  ( 36.86361269976527666, -285.7368702992679346, -273.8409634762059568 ) ) ;
#56983=CARTESIAN_POINT ( 'NONE',  ( -3.455197931748154261, -292.6047140793157268, -337.2836856663037111 ) ) ;
#56984=CARTESIAN_POINT ( 'NONE',  ( -85.67825976110560759, -282.1872209888519478, -329.4058870458297292 ) ) ;
#56985=CARTESIAN_POINT ( 'NONE',  ( -101.5174171983701967, -280.6459334508145389, -233.9205121687215865 ) ) ;
#56986=CARTESIAN_POINT ( 'NONE',  ( -87.50158432319115320, -286.5757132716646538, -212.3944682455413897 ) ) ;
#56987=CARTESIAN_POINT ( 'NONE',  ( 19.38730561538277897, -279.0973403998557387, -219.7866858338066720 ) ) ;
#56988=CARTESIAN_POINT ( 'NONE',  ( 33.70108727723620490, -287.7736599881156963, -287.1516616808103777 ) ) ;
#56989=CARTESIAN_POINT ( 'NONE',  ( -105.8094356715702560, -279.6195923458071206, -297.3341434989458776 ) ) ;
#56990=CARTESIAN_POINT ( 'NONE',  ( -96.54237104610450615, -279.9552479132331086, -227.3741165733673029 ) ) ;
#56991=CARTESIAN_POINT ( 'NONE',  ( 13.12619323610478261, -288.7327171141691906, -214.3322335487033854 ) ) ;
#56993=CARTESIAN_POINT ( 'NONE',  ( -85.21476000888939950, -297.2447833527709804, -210.0521622451851442 ) ) ;
#56994=CARTESIAN_POINT ( 'NONE',  ( -37.24104840482309697, -291.0307759980611308, -345.0058544116742496 ) ) ;
#56996=CARTESIAN_POINT ( 'NONE',  ( -111.2586520408596868, -286.6233781216988064, -305.9938812882205070 ) ) ;
#56998=CARTESIAN_POINT ( 'NONE',  ( -35.54153654152194264, -272.0745038759882277, -195.2031888215580580 ) ) ;
#57000=CARTESIAN_POINT ( 'NONE',  ( 34.72310501556402329, -292.2692172039432421, -295.2836283584013017 ) ) ;
#57001=CARTESIAN_POINT ( 'NONE',  ( -110.4356889987182768, -296.0813631412486870, -268.7252675560291095 ) ) ;
#57002=CARTESIAN_POINT ( 'NONE',  ( -33.21904697282409558, -287.6249900601071090, -196.7328961683710133 ) ) ;
#57003=CARTESIAN_POINT ( 'NONE',  ( 36.03439874259679954, -283.1812574738265766, -260.2895952477425112 ) ) ;
#57004=CARTESIAN_POINT ( 'NONE',  ( -75.35467898774608386, -290.9739855493204459, -336.6455032572121127 ) ) ;
#57005=CARTESIAN_POINT ( 'NONE',  ( -75.40371254366711185, -290.8639050383438871, -336.7281390379810091 ) ) ;
#57006=CARTESIAN_POINT ( 'NONE',  ( -103.5244373229910479, -286.0830144231047711, -305.7539570117792778 ) ) ;
#57007=CARTESIAN_POINT ( 'NONE',  ( -56.92197987009077309, -277.4644614284491126, -344.8850404908887981 ) ) ;
#57009=CARTESIAN_POINT ( 'NONE',  ( 10.27159629921781026, -292.4814568221828495, -329.0995434034642244 ) ) ;
#57010=CARTESIAN_POINT ( 'NONE',  ( -6.228421261166688261, -280.2830642313593899, -199.9127353148523412 ) ) ;
#57011=CARTESIAN_POINT ( 'NONE',  ( -110.3487966584650053, -274.5905835462723985, -256.6384011743670044 ) ) ;
#57012=CARTESIAN_POINT ( 'NONE',  ( 31.95455697924148097, -295.6233781216988632, -236.9535640164627637 ) ) ;
#57013=CARTESIAN_POINT ( 'NONE',  ( 2.944996183118116395, -274.7595557134114870, -334.8509593743912092 ) ) ;
#57015=CARTESIAN_POINT ( 'NONE',  ( 35.62706769095613879, -281.1083151865499303, -274.0417924396392095 ) ) ;
#57016=CARTESIAN_POINT ( 'NONE',  ( -113.9873588511679969, -279.7414350433387540, -271.6172805357961124 ) ) ;
#57017=CARTESIAN_POINT ( 'NONE',  ( -75.53183120188381849, -298.9575618885363610, -207.3982246520323827 ) ) ;
#57018=CARTESIAN_POINT ( 'NONE',  ( -78.38650515326199297, -284.5728664480191696, -205.4909076155248613 ) ) ;
#57019=CARTESIAN_POINT ( 'NONE',  ( -110.2792174653791335, -292.4797049607450390, -257.4945063852299540 ) ) ;
#57020=CARTESIAN_POINT ( 'NONE',  ( -64.63279250055867919, -275.3018531292676130, -199.2018976324963546 ) ) ;
#57021=CARTESIAN_POINT ( 'NONE',  ( -41.18486414913537885, -275.3200356171304861, -193.8989300784495526 ) ) ;
#57023=CARTESIAN_POINT ( 'NONE',  ( -25.90265132006070559, -296.9062861093387937, -344.3149994667273859 ) ) ;
#57024=CARTESIAN_POINT ( 'NONE',  ( -68.57212797090788570, -281.4633582659103013, -338.3661825511899224 ) ) ;
#57025=CARTESIAN_POINT ( 'NONE',  ( -111.6112754635759075, -290.4730434448304095, -250.0682234348522854 ) ) ;
#57026=CARTESIAN_POINT ( 'NONE',  ( 26.77580129805163267, -274.0861768400902747, -308.5814373393323535 ) ) ;
#57027=CARTESIAN_POINT ( 'NONE',  ( 22.35232823133723912, -288.5115964331699274, -222.9793381090060791 ) ) ;
#57028=CARTESIAN_POINT ( 'NONE',  ( -90.97599986096025759, -290.1882495241550828, -220.3666878367873210 ) ) ;
#57030=CARTESIAN_POINT ( 'NONE',  ( -112.7812274638141048, -288.9738315548914898, -282.5054174105057427 ) ) ;
#57031=CARTESIAN_POINT ( 'NONE',  ( -77.26316839752735177, -291.1671353052126960, -209.2189569319506575 ) ) ;
#57033=CARTESIAN_POINT ( 'NONE',  ( 26.09391856048089053, -288.0610159307652225, -227.2399295133388648 ) ) ;
#57034=CARTESIAN_POINT ( 'NONE',  ( 13.74915395457545664, -276.6453514654967307, -322.6025318019650854 ) ) ;
#57035=CARTESIAN_POINT ( 'NONE',  ( -22.17218938640405312, -293.7825439556069114, -345.5367686465120869 ) ) ;
#57036=CARTESIAN_POINT ( 'NONE',  ( -71.68576130064883500, -284.1454699585555659, -339.1637214888811513 ) ) ;
#57037=CARTESIAN_POINT ( 'NONE',  ( -69.78779512738151425, -285.9698201995951194, -200.5399141243469217 ) ) ;
#57038=CARTESIAN_POINT ( 'NONE',  ( -58.95034025699933267, -283.6727034005659220, -340.1649311593427569 ) ) ;
#57039=CARTESIAN_POINT ( 'NONE',  ( -22.29584452022010410, -108.1748762211270076, -362.7363045332584193 ) ) ;
#57040=CARTESIAN_POINT ( 'NONE',  ( -32.08198064645461756, -123.8691969543307891, -363.6799844872283529 ) ) ;
#57041=CARTESIAN_POINT ( 'NONE',  ( 24.66845159430726753, -23.60273429576747972, -341.5102311320878812 ) ) ;
#57042=CARTESIAN_POINT ( 'NONE',  ( -31.31624232178432266, -273.3273285971770292, -197.4355088390831554 ) ) ;
#57043=CARTESIAN_POINT ( 'NONE',  ( -38.07170090988125821, -272.9631189479677005, -197.0556395139649055 ) ) ;
#57044=CARTESIAN_POINT ( 'NONE',  ( -107.1132046348760412, -295.6444724115103213, -302.7874045709687039 ) ) ;
#57045=CARTESIAN_POINT ( 'NONE',  ( -101.4239464694510815, -254.8757987455171303, -324.3748491368189093 ) ) ;
#57047=CARTESIAN_POINT ( 'NONE',  ( -76.16792024306317899, -272.2298729070964214, -204.3770549805997803 ) ) ;
#57048=CARTESIAN_POINT ( 'NONE',  ( -93.69731465116937841, -299.0891298078469731, -222.0206491791082613 ) ) ;
#57050=CARTESIAN_POINT ( 'NONE',  ( 3.905138949092443301, -289.7993641071265074, -331.2496380871870088 ) ) ;
#57051=CARTESIAN_POINT ( 'NONE',  ( -108.7316297353748240, -291.8514498473621757, -253.6418770121819364 ) ) ;
#57053=CARTESIAN_POINT ( 'NONE',  ( -82.84078776837078806, -298.3883985450590330, -208.4674559683344910 ) ) ;
#57054=CARTESIAN_POINT ( 'NONE',  ( 27.08768995313700856, -288.5150020839810736, -304.9193862970209352 ) ) ;
#57055=CARTESIAN_POINT ( 'NONE',  ( 6.530208131676044303, -295.2756834791700271, -333.5085562059158519 ) ) ;
#57056=CARTESIAN_POINT ( 'NONE',  ( -81.83100278750610812, -296.1323502263370528, -333.1974273120356429 ) ) ;
#57057=CARTESIAN_POINT ( 'NONE',  ( 34.21606884034724771, -293.5283579228146777, -255.9220839154837108 ) ) ;
#57059=CARTESIAN_POINT ( 'NONE',  ( 37.88121963091056443, -277.3746875442321311, -262.7015421438641738 ) ) ;
#57061=CARTESIAN_POINT ( 'NONE',  ( -68.64174411570809298, -279.1593725660400196, -200.0627906718582381 ) ) ;
#57062=CARTESIAN_POINT ( 'NONE',  ( 35.93446212157289210, -276.5093973065011710, -271.5769497896921507 ) ) ;
#57063=CARTESIAN_POINT ( 'NONE',  ( -46.77767594461364098, -275.6940480370619184, -194.9626009363000207 ) ) ;
#57064=CARTESIAN_POINT ( 'NONE',  ( 37.68233627622525006, -273.4752696502167169, -262.7716176065841296 ) ) ;
#57065=CARTESIAN_POINT ( 'NONE',  ( -34.48323562599132686, -298.7402805562511503, -197.2588576385242050 ) ) ;
#57066=CARTESIAN_POINT ( 'NONE',  ( -73.60847255458759264, -294.1183427976135363, -334.3931110439744430 ) ) ;
#57068=CARTESIAN_POINT ( 'NONE',  ( -112.9368912412941341, -279.2245402869689315, -255.9765108116061185 ) ) ;
#57069=CARTESIAN_POINT ( 'NONE',  ( -1.468378563068700071, -276.7293780571827710, -333.9958696484717393 ) ) ;
#57070=CARTESIAN_POINT ( 'NONE',  ( 24.31583636898643874, -285.6314728445236142, -225.0660137560103067 ) ) ;
#57071=CARTESIAN_POINT ( 'NONE',  ( -4.439390663982942797, -300.4632727336159519, -195.1832562283304071 ) ) ;
#57073=CARTESIAN_POINT ( 'NONE',  ( 19.64740117131388786, -286.1019006774488957, -224.4626861561665976 ) ) ;
#57074=CARTESIAN_POINT ( 'NONE',  ( -36.98120204125686428, -278.2965856733780470, -196.3486591815759255 ) ) ;
#57075=CARTESIAN_POINT ( 'NONE',  ( -110.5503501736334044, -277.2310611430731910, -262.3993772893183518 ) ) ;
#57076=CARTESIAN_POINT ( 'NONE',  ( -39.26865653978450865, -285.0764670791407411, -345.3489154689093539 ) ) ;
#57077=CARTESIAN_POINT ( 'NONE',  ( -9.825337146746806027, -277.8896722950271965, -338.4187172147080673 ) ) ;
#57079=CARTESIAN_POINT ( 'NONE',  ( -7.000189698666798854, -274.8993490968689457, -340.0412934062130716 ) ) ;
#57080=CARTESIAN_POINT ( 'NONE',  ( -46.19934488342533996, -274.5882315184521758, -197.7978021994498192 ) ) ;
#57081=CARTESIAN_POINT ( 'NONE',  ( 37.70065986253945312, -283.6182716926127227, -275.5093361847587516 ) ) ;
#57083=CARTESIAN_POINT ( 'NONE',  ( -6.197271525055271901, -290.5662769388397351, -339.2039735899903121 ) ) ;
#57084=CARTESIAN_POINT ( 'NONE',  ( 34.38626963407741499, -291.2690379094027548, -248.4064131804255737 ) ) ;
#57086=CARTESIAN_POINT ( 'NONE',  ( -46.22187263709554372, -272.6219611984311086, -197.4064333237768381 ) ) ;
#57087=CARTESIAN_POINT ( 'NONE',  ( 11.76535650949521994, -290.8818022956375557, -214.6205859784895154 ) ) ;
#57088=CARTESIAN_POINT ( 'NONE',  ( -68.16629546550866792, -198.4621125041185792, -363.1570911012638021 ) ) ;
#57090=CARTESIAN_POINT ( 'NONE',  ( -70.35677490696174630, -287.9592243844340373, -339.1701881515262471 ) ) ;
#57091=CARTESIAN_POINT ( 'NONE',  ( -69.33776954806731396, -285.0804659685678075, -336.8783928411505713 ) ) ;
#57092=CARTESIAN_POINT ( 'NONE',  ( -1.428432174047877146, -284.7615873765060428, -203.3968648305780675 ) ) ;
#57093=CARTESIAN_POINT ( 'NONE',  ( -76.42480920467323813, -285.0109203883594660, -332.7742844648213350 ) ) ;
#57094=CARTESIAN_POINT ( 'NONE',  ( -71.47517675281146410, -284.3180443054658895, -335.0720714670007396 ) ) ;
#57095=CARTESIAN_POINT ( 'NONE',  ( -72.68506834579171993, -293.5664524536089743, -203.7939000390738613 ) ) ;
#57096=CARTESIAN_POINT ( 'NONE',  ( 27.28386481134897679, -273.1100762290441821, -231.1094067317442864 ) ) ;
#57097=CARTESIAN_POINT ( 'NONE',  ( -67.53126134894574761, -274.0000681242288465, -199.5491508804911120 ) ) ;
#57098=CARTESIAN_POINT ( 'NONE',  ( -109.4158251411403313, -288.3395239986521688, -293.2177928206025967 ) ) ;
#57099=CARTESIAN_POINT ( 'NONE',  ( -6.574700718552085377, -276.6592058320854903, -340.9614332825877341 ) ) ;
#57100=CARTESIAN_POINT ( 'NONE',  ( 4.764527462724890583, -296.4602639153259815, -331.9964357683143135 ) ) ;
#57102=CARTESIAN_POINT ( 'NONE',  ( 10.64812456238590066, -296.9090924074130271, -330.4860931364851808 ) ) ;
#57103=CARTESIAN_POINT ( 'NONE',  ( -105.0453732086373719, -283.6197080951067733, -241.6391943592855114 ) ) ;
#57104=CARTESIAN_POINT ( 'NONE',  ( 0.3904103032349110491, -278.5542552050746963, -205.4846325138206851 ) ) ;
#57106=CARTESIAN_POINT ( 'NONE',  ( -96.38714683788903415, -271.6871196828031998, -222.0050020251756564 ) ) ;
#57107=CARTESIAN_POINT ( 'NONE',  ( -72.89883278356163032, -276.8850848172081101, -334.2471339079709196 ) ) ;
#57108=CARTESIAN_POINT ( 'NONE',  ( 23.14606162351636343, -294.4908024231062882, -228.2444928478107045 ) ) ;
#57109=CARTESIAN_POINT ( 'NONE',  ( -1.150794669299052497, -293.4862282978351118, -206.6784984058583632 ) ) ;
#57110=CARTESIAN_POINT ( 'NONE',  ( -44.73121370613633729, -296.4588562552970643, -346.5633340154544157 ) ) ;
#57111=CARTESIAN_POINT ( 'NONE',  ( -109.2754964653054799, -296.5494565336858841, -257.9301506416070993 ) ) ;
#57112=CARTESIAN_POINT ( 'NONE',  ( -23.38877885651763222, -290.8740657422976597, -344.1049187710933097 ) ) ;
#57113=CARTESIAN_POINT ( 'NONE',  ( -27.36999740024758410, -283.0955926159798537, -346.7660682773487224 ) ) ;
#57114=CARTESIAN_POINT ( 'NONE',  ( -82.81943784833634936, -271.5776928330944315, -209.6977741619279811 ) ) ;
#57115=CARTESIAN_POINT ( 'NONE',  ( 18.35296504267913420, -286.6577035833771561, -217.1136988799782443 ) ) ;
#57116=CARTESIAN_POINT ( 'NONE',  ( -72.93573347164384302, -281.5579298806165411, -204.7492928676206247 ) ) ;
#57117=CARTESIAN_POINT ( 'NONE',  ( -95.94705082875732671, -284.2254147920054947, -226.4427696760492097 ) ) ;
#57118=CARTESIAN_POINT ( 'NONE',  ( -10.30860769527706289, -286.6991876892269033, -340.3197669299837003 ) ) ;
#57119=CARTESIAN_POINT ( 'NONE',  ( 89.65909921107042635, 79.73535476480827811, -300.8268380169218972 ) ) ;
#57120=CARTESIAN_POINT ( 'NONE',  ( -11.99475968347147692, -285.8988215653403131, -201.8372458521104420 ) ) ;
#57121=CARTESIAN_POINT ( 'NONE',  ( -10.77218981492375072, -283.6553643448311277, -342.4376012753236296 ) ) ;
#57122=CARTESIAN_POINT ( 'NONE',  ( -112.9382155646799930, -289.7782652271950496, -257.0199386058425830 ) ) ;
#57123=CARTESIAN_POINT ( 'NONE',  ( -107.7809798661091492, -280.5255459192690637, -241.2965642502736330 ) ) ;
#57124=CARTESIAN_POINT ( 'NONE',  ( -84.27768560191996983, -280.7372519531672310, -209.8762566701305445 ) ) ;
#57125=CARTESIAN_POINT ( 'NONE',  ( 26.85404104593239083, -281.8596809207245997, -305.1160718683655091 ) ) ;
#57126=CARTESIAN_POINT ( 'NONE',  ( 16.87543678902525457, -276.8239737314597733, -218.4641316652456737 ) ) ;
#57127=CARTESIAN_POINT ( 'NONE',  ( -61.59156506239160223, -295.3585754478501713, -343.4986196502385383 ) ) ;
#57128=CARTESIAN_POINT ( 'NONE',  ( -70.73033779678549138, -287.5148011609784362, -337.1364013218289415 ) ) ;
#57129=CARTESIAN_POINT ( 'NONE',  ( -2.440602311976399541, -294.1061240800694918, -202.6091071351043809 ) ) ;
#57130=CARTESIAN_POINT ( 'NONE',  ( -108.8965749324479333, -295.2630727645437219, -286.3024468618982041 ) ) ;
#57132=CARTESIAN_POINT ( 'NONE',  ( -18.34500948516543062, -284.7257828497566834, -342.3898341017015241 ) ) ;
#57133=CARTESIAN_POINT ( 'NONE',  ( -109.7566344058575964, -296.3477331068804688, -260.5897039882700028 ) ) ;
#57134=CARTESIAN_POINT ( 'NONE',  ( 39.29847969715857658, -294.6668356569264802, -273.1495485930986433 ) ) ;
#57135=CARTESIAN_POINT ( 'NONE',  ( -36.18360817194103163, -283.6886669524637341, -343.4538774841473128 ) ) ;
#57137=CARTESIAN_POINT ( 'NONE',  ( -36.92892426766344016, -273.1159871622386959, -193.5845085195130366 ) ) ;
#57138=CARTESIAN_POINT ( 'NONE',  ( -51.65818546520302590, -289.8821002412654479, -345.9147481658728793 ) ) ;
#57139=CARTESIAN_POINT ( 'NONE',  ( -3.466709903770705203, -280.7494329135404314, -338.1456643307538457 ) ) ;
#57140=CARTESIAN_POINT ( 'NONE',  ( -107.2430110538742554, -291.2994238896230286, -237.9920331185965097 ) ) ;
#57141=CARTESIAN_POINT ( 'NONE',  ( 12.17325497759521546, -288.6739031020745756, -324.0987852835651779 ) ) ;
#57144=CARTESIAN_POINT ( 'NONE',  ( 121.4028569870072971, 147.5259734495768669, -260.2187139711599002 ) ) ;
#57145=CARTESIAN_POINT ( 'NONE',  ( -110.4542110544635705, -270.2666405000204009, -253.6410175316879361 ) ) ;
#57146=CARTESIAN_POINT ( 'NONE',  ( -108.3312468908004860, -277.5157186597799068, -288.1070286343262410 ) ) ;
#57148=CARTESIAN_POINT ( 'NONE',  ( -54.55207517852110755, -278.7462307273775650, -199.0484115112007544 ) ) ;
#57149=CARTESIAN_POINT ( 'NONE',  ( 37.61529595931217074, -274.9989619022424563, -252.7768409693519800 ) ) ;
#57150=CARTESIAN_POINT ( 'NONE',  ( 123.2339866187729598, 147.3305397618446761, -261.4581277174236220 ) ) ;
#57152=CARTESIAN_POINT ( 'NONE',  ( -68.41615132926648357, -278.2265983074422024, -200.5400767411933600 ) ) ;
#57153=CARTESIAN_POINT ( 'NONE',  ( -79.32202510925571914, -281.6420802453622514, -332.0822579186136636 ) ) ;
#57154=CARTESIAN_POINT ( 'NONE',  ( -85.73252688891574280, -297.4716991039567802, -328.9469686353702969 ) ) ;
#57155=CARTESIAN_POINT ( 'NONE',  ( 33.70613836740976410, -293.8193092850265202, -253.2726355837552887 ) ) ;
#57157=CARTESIAN_POINT ( 'NONE',  ( -105.5771151798270751, -288.8724559585137399, -297.7956129173536510 ) ) ;
#57158=CARTESIAN_POINT ( 'NONE',  ( -35.53450855500613415, -274.7256487033095596, -193.4711760317047720 ) ) ;
#57159=CARTESIAN_POINT ( 'NONE',  ( -94.61271035972472987, -273.1909261468162526, -225.0948900963422545 ) ) ;
#57163=B_SPLINE_CURVE_WITH_KNOTS ( 'NONE', 3,
 ( #36804, #21202, #65725, #37716, #836, #66622, #30634, #58600, #88383, #75583, #52402, #38180, #38657, #16425, #45277, #32959 ),
 .UNSPECIFIED., .F., .F.,
 ( 4, 2, 2, 2, 2, 2, 2, 4 ),
 ( 0.1790892544726606084, 0.2192030976635781225, 0.2593169408544956367, 0.2994307840454131231, 0.3395446272363306095, 0.3796584704272480959, 0.4197723136181656378, 0.5000000000000000000 ),
 .UNSPECIFIED. ) ;
#57165=CARTESIAN_POINT ( 'NONE',  ( -30.24609430240859353, -281.2235581765413599, -197.3456372872051929 ) ) ;
#57166=CARTESIAN_POINT ( 'NONE',  ( -28.36722641797974731, -281.9245260274670954, -194.8533604755647559 ) ) ;
#57167=CARTESIAN_POINT ( 'NONE',  ( -89.06894425974725493, -282.8599196068099104, -322.2753491389266856 ) ) ;
#57168=CARTESIAN_POINT ( 'NONE',  ( 23.10574395892109578, -282.8205770558491281, -227.2685201845750100 ) ) ;
#57169=CARTESIAN_POINT ( 'NONE',  ( 12.19962523608213090, -274.8280794452312534, -324.9864160017370978 ) ) ;
#57172=CARTESIAN_POINT ( 'NONE',  ( -110.5097548597353239, -279.0573914041060561, -293.9971085231694019 ) ) ;
#57174=ORIENTED_EDGE ( 'NONE', *, *, #72721, .F. ) ;
#57176=CARTESIAN_POINT ( 'NONE',  ( -47.01960340857906573, -285.1543968441169454, -345.0922693801278456 ) ) ;
#57177=CARTESIAN_POINT ( 'NONE',  ( 21.94154536604866834, -292.1506265979649584, -227.4667592680269195 ) ) ;
#57178=CARTESIAN_POINT ( 'NONE',  ( 32.76853770057452664, -287.3047797470836144, -301.9501562377100186 ) ) ;
#57179=CARTESIAN_POINT ( 'NONE',  ( -62.89193534206738434, -283.9548899151191677, -200.8431004805752593 ) ) ;
#57180=CARTESIAN_POINT ( 'NONE',  ( -105.1333447811755377, -283.5096275338648297, -241.6003774355187375 ) ) ;
#57181=CARTESIAN_POINT ( 'NONE',  ( -26.34618162670978947, -287.1502995099515374, -343.6048999761332539 ) ) ;
#57182=CARTESIAN_POINT ( 'NONE',  ( -37.52619258083087317, -284.2596254218029799, -343.7704570217542823 ) ) ;
#57183=CARTESIAN_POINT ( 'NONE',  ( 16.66751951071931970, -272.8198321970713209, -218.2480451313527396 ) ) ;
#57184=CARTESIAN_POINT ( 'NONE',  ( -113.1105788464700623, -282.8497328983733041, -278.4554019020054625 ) ) ;
#57185=CARTESIAN_POINT ( 'NONE',  ( -36.27661821145474619, -297.0389920560507448, -345.3663223176694146 ) ) ;
#57186=CARTESIAN_POINT ( 'NONE',  ( -67.73552806259097281, -283.6541095752592696, -201.5994054247314580 ) ) ;
#57187=CARTESIAN_POINT ( 'NONE',  ( -83.59559592967119102, -280.3410856909468976, -213.5153204770480215 ) ) ;
#57191=CARTESIAN_POINT ( 'NONE',  ( 28.33535374304726417, -295.9679175910864615, -307.8277992328399364 ) ) ;
#57192=CARTESIAN_POINT ( 'NONE',  ( -110.7268525702525892, -276.3532372884859569, -285.8407837970616470 ) ) ;
#57193=CARTESIAN_POINT ( 'NONE',  ( -103.0723992339431447, -290.2709716151322823, -230.4636555132805995 ) ) ;
#57194=CARTESIAN_POINT ( 'NONE',  ( 16.73158051365991739, -292.6661275954513144, -320.5858204322466349 ) ) ;
#57195=CARTESIAN_POINT ( 'NONE',  ( -43.77769788857359856, -278.6540795477220058, -197.0997434678387208 ) ) ;
#57196=CARTESIAN_POINT ( 'NONE',  ( -103.2951584642906511, -271.0939850566395535, -235.7320767071639693 ) ) ;
#57197=CARTESIAN_POINT ( 'NONE',  ( -93.82955868861657223, -292.5300387966336757, -223.3269435335836306 ) ) ;
#57198=CARTESIAN_POINT ( 'NONE',  ( -85.28047601435906699, -286.1948066931273615, -330.5268031993605859 ) ) ;
#57199=CARTESIAN_POINT ( 'NONE',  ( -11.31208035220853780, -293.1990793112764209, -342.1469892098484138 ) ) ;
#57200=CARTESIAN_POINT ( 'NONE',  ( -71.52541129064096026, -291.1116395513638508, -335.7811601952328147 ) ) ;
#57201=CARTESIAN_POINT ( 'NONE',  ( -34.96929491566408643, -290.3213960246039846, -194.3985150574085878 ) ) ;
#57202=CARTESIAN_POINT ( 'NONE',  ( -42.68875334143204014, -290.5460647466658770, -343.8068434839705674 ) ) ;
#57204=CARTESIAN_POINT ( 'NONE',  ( -5.713389437453334274, -289.4280564095175237, -336.3327155866107887 ) ) ;
#57205=FACE_OUTER_BOUND ( 'NONE', #18092, .T. ) ;
#57206=CARTESIAN_POINT ( 'NONE',  ( -113.7152737123392825, -291.6745858203403827, -276.9348716747363710 ) ) ;
#57207=CARTESIAN_POINT ( 'NONE',  ( 18.54631275297971271, -280.2743613275927714, -320.9838113474575039 ) ) ;
#57208=CARTESIAN_POINT ( 'NONE',  ( -108.6627219916117895, -290.3460958610340299, -285.9855972731699012 ) ) ;
#57209=CARTESIAN_POINT ( 'NONE',  ( -59.30017208588333233, -280.1087202447411073, -196.5805663396793932 ) ) ;
#57210=CARTESIAN_POINT ( 'NONE',  ( 4.530635706834868159, -282.1707915009040448, -335.0186348953547508 ) ) ;
#57211=CARTESIAN_POINT ( 'NONE',  ( 21.92257918866998523, -286.1823452636505749, -316.3465169579442886 ) ) ;
#57213=CARTESIAN_POINT ( 'NONE',  ( 14.77526791730137923, -280.4484569966114123, -323.2982713932576075 ) ) ;
#57214=CARTESIAN_POINT ( 'NONE',  ( -102.2952847834866930, -283.0536750571794755, -232.7607990155565574 ) ) ;
#57217=CARTESIAN_POINT ( 'NONE',  ( -108.0215781079693897, -276.6634829867090843, -299.1198140572902844 ) ) ;
#57218=CARTESIAN_POINT ( 'NONE',  ( -12.78960523482254885, -285.2843270950392593, -197.7065438278079910 ) ) ;
#57219=CARTESIAN_POINT ( 'NONE',  ( -27.27806132797662642, -274.9860188879577549, -197.8440815844289205 ) ) ;
#57220=CARTESIAN_POINT ( 'NONE',  ( 114.7448031289451222, -299.5541904835127980, -192.4214616598467273 ) ) ;
#57221=CARTESIAN_POINT ( 'NONE',  ( -47.12041845921879002, -293.5259977270851550, -197.2118385478385676 ) ) ;
#57222=CARTESIAN_POINT ( 'NONE',  ( 37.90863464353293466, -276.8092866274533321, -257.0202020678862027 ) ) ;
#57223=CARTESIAN_POINT ( 'NONE',  ( -70.46618380594966879, -277.1681781447261415, -335.4368897254521471 ) ) ;
#57224=CARTESIAN_POINT ( 'NONE',  ( -111.9950936832419472, -290.9554713978622544, -251.4434639793408053 ) ) ;
#57225=CARTESIAN_POINT ( 'NONE',  ( 36.84559428790554847, -279.4492764055048042, -256.0237699762428178 ) ) ;
#57226=CARTESIAN_POINT ( 'NONE',  ( 11.12043451956602169, -292.5350696141254048, -210.4558940542265191 ) ) ;
#57227=CARTESIAN_POINT ( 'NONE',  ( -83.96965594986329506, -290.4516713222828912, -213.8877421027370076 ) ) ;
#57228=CARTESIAN_POINT ( 'NONE',  ( 16.11761735759916192, -292.2941826330477397, -323.0382098874331973 ) ) ;
#57231=CARTESIAN_POINT ( 'NONE',  ( 21.85825109088264639, -292.4610618157944941, -227.5221553818784059 ) ) ;
#57233=CARTESIAN_POINT ( 'NONE',  ( -6.941161984400256557, -271.9809262143061233, -207.3071070584150277 ) ) ;
#57234=CARTESIAN_POINT ( 'NONE',  ( -95.41138479463613464, -294.9306069910667247, -320.5680093043957299 ) ) ;
#57235=CARTESIAN_POINT ( 'NONE',  ( -109.5176107783252917, -286.1894963474462656, -244.9852200883260593 ) ) ;
#57236=CARTESIAN_POINT ( 'NONE',  ( -27.83445044074651165, -286.0095681809751227, -197.9828601430970707 ) ) ;
#57237=CARTESIAN_POINT ( 'NONE',  ( 36.27851160155952925, -277.0163323146715015, -266.0795742938309445 ) ) ;
#57238=CARTESIAN_POINT ( 'NONE',  ( -7.350068831619500642, -292.6770215717642145, -338.7295805699538391 ) ) ;
#57239=CARTESIAN_POINT ( 'NONE',  ( -108.4389337298712519, -298.5806465622432029, -249.7903282865496521 ) ) ;
#57240=CARTESIAN_POINT ( 'NONE',  ( 36.04020802804998169, -274.3274940996295754, -268.8691196571160162 ) ) ;
#57243=CARTESIAN_POINT ( 'NONE',  ( -66.92023900696986516, -295.0960279561686548, -341.4446789513162912 ) ) ;
#57244=CARTESIAN_POINT ( 'NONE',  ( 31.83220830565329607, -289.8347671409260329, -298.0008877410383548 ) ) ;
#57246=CARTESIAN_POINT ( 'NONE',  ( -100.8877902063416485, -274.3247652036166073, -227.4892895565202480 ) ) ;
#57247=CARTESIAN_POINT ( 'NONE',  ( 31.49817532150609622, -288.5305974993274276, -294.9571383140427656 ) ) ;
#57250=CARTESIAN_POINT ( 'NONE',  ( -69.85178790822799044, -278.6932197091731496, -200.8060342518697041 ) ) ;
#57251=CARTESIAN_POINT ( 'NONE',  ( -64.22277405604366152, -296.0452728255502279, -342.4077740534941086 ) ) ;
#57252=CARTESIAN_POINT ( 'NONE',  ( -54.24939633010384910, -287.4065000605688738, -344.2691044333760715 ) ) ;
#57253=CARTESIAN_POINT ( 'NONE',  ( -61.58088049430824640, -295.6918029353748807, -343.4798708562101979 ) ) ;
#57254=CARTESIAN_POINT ( 'NONE',  ( 20.54256203885854504, -294.5119443429359762, -314.8956309882918845 ) ) ;
#57257=CARTESIAN_POINT ( 'NONE',  ( 37.34089866539330416, -288.8738484990258257, -254.6385142663085617 ) ) ;
#57258=CARTESIAN_POINT ( 'NONE',  ( -55.56934967048407970, -289.3380690714490129, -190.3538533559490702 ) ) ;
#57260=CARTESIAN_POINT ( 'NONE',  ( -103.3198664937667530, -278.4176495018903665, -230.7583048782927051 ) ) ;
#57261=CARTESIAN_POINT ( 'NONE',  ( -7.746323770853920543, -284.6635433926473411, -339.0935130160386279 ) ) ;
#57262=CARTESIAN_POINT ( 'NONE',  ( -106.1406452522187323, -283.5567514552673174, -237.1148935189554550 ) ) ;
#57263=CARTESIAN_POINT ( 'NONE',  ( -51.03998138331096612, -287.3082637710973586, -343.5826057218839651 ) ) ;
#57264=CARTESIAN_POINT ( 'NONE',  ( -17.65564194824074562, -278.6612672932710097, -343.5237080903923470 ) ) ;
#57266=CARTESIAN_POINT ( 'NONE',  ( -74.01327642203473545, -277.5540697996185600, -333.4816019169909964 ) ) ;
#57267=CARTESIAN_POINT ( 'NONE',  ( -72.17098014583973509, -278.9270496204223377, -206.0897097061223917 ) ) ;
#57268=CARTESIAN_POINT ( 'NONE',  ( -46.85633122383234905, -275.0136878641828844, -194.2627322943047261 ) ) ;
#57269=CARTESIAN_POINT ( 'NONE',  ( -113.6468991498996104, -277.4391573486000766, -263.0365485044620755 ) ) ;
#57270=CARTESIAN_POINT ( 'NONE',  ( 63.23836714137711112, 47.77599596953215411, -316.5090406242446761 ) ) ;
#57271=CARTESIAN_POINT ( 'NONE',  ( -67.45441980011311500, -274.6079407048925418, -199.7491903263003792 ) ) ;
#57273=CARTESIAN_POINT ( 'NONE',  ( -15.04246470041792705, -299.7514418032953358, -193.9450587403573820 ) ) ;
#57274=CARTESIAN_POINT ( 'NONE',  ( -54.49178911615187815, -288.3376638359845856, -195.3683826091709363 ) ) ;
#57277=CARTESIAN_POINT ( 'NONE',  ( 82.65162136640255142, -299.3405935325396854, -192.8643928579782596 ) ) ;
#57278=CARTESIAN_POINT ( 'NONE',  ( -46.77822599613994470, -287.0093449685113001, -197.6108968973923652 ) ) ;
#57279=CARTESIAN_POINT ( 'NONE',  ( 0.9908731529661984894, -288.3164198519621095, -204.7366259479212260 ) ) ;
#57280=CARTESIAN_POINT ( 'NONE',  ( 22.03965603196966683, -287.4959265442595324, -312.9961647043861603 ) ) ;
#57281=CARTESIAN_POINT ( 'NONE',  ( -114.1473530375246241, -283.9928917890878211, -275.7072527118373273 ) ) ;
#57282=CARTESIAN_POINT ( 'NONE',  ( -74.89551508447735273, -277.9433878448719497, -206.7716755640965687 ) ) ;
#57283=CARTESIAN_POINT ( 'NONE',  ( -46.90711468948353513, -287.7899637299429969, -196.6931233092008426 ) ) ;
#57284=CARTESIAN_POINT ( 'NONE',  ( 33.62192456028797949, -280.2922032504346816, -290.2324975170747052 ) ) ;
#57285=CARTESIAN_POINT ( 'NONE',  ( -48.66742310038758035, -278.5144238102573695, -343.0280814630534678 ) ) ;
#57286=CARTESIAN_POINT ( 'NONE',  ( 28.08840541023383253, -276.4863082384095492, -302.9850296949877020 ) ) ;
#57287=CARTESIAN_POINT ( 'NONE',  ( -71.74197864103589950, -288.2915764510409531, -338.8054717186547578 ) ) ;
#57288=CARTESIAN_POINT ( 'NONE',  ( -24.55037457845733329, -283.6958537371342572, -346.1814783090250671 ) ) ;
#57289=CARTESIAN_POINT ( 'NONE',  ( -107.8722291171190193, -285.4382007472626128, -239.4874949684683827 ) ) ;
#57290=CARTESIAN_POINT ( 'NONE',  ( -24.87847801729734698, -280.3822679026047808, -198.4329030797603650 ) ) ;
#57293=DIRECTION ( 'NONE',  ( 1.000000000000000000, 0.000000000000000000, 0.000000000000000000 ) ) ;
#57294=CARTESIAN_POINT ( 'NONE',  ( -70.08347964180700274, -291.3392148065165088, -338.7001921549091890 ) ) ;
#57295=CARTESIAN_POINT ( 'NONE',  ( -93.24398708872134023, -288.5194553016125951, -322.6699744567048356 ) ) ;
#57296=CARTESIAN_POINT ( 'NONE',  ( -109.8138290549240708, -271.7541084127307158, -259.4698463676803613 ) ) ;
#57297=CARTESIAN_POINT ( 'NONE',  ( 34.35345792672862331, -293.2534736440766210, -298.1661013100909372 ) ) ;
#57298=CARTESIAN_POINT ( 'NONE',  ( -45.45785259689345992, -287.6367268037397480, -343.6061575484424111 ) ) ;
#57299=CARTESIAN_POINT ( 'NONE',  ( 30.79730872466732450, -291.4078086117562520, -241.3326806734435763 ) ) ;
#57300=CARTESIAN_POINT ( 'NONE',  ( 34.09324062552919088, -288.5353403252199200, -253.4492162859894790 ) ) ;
#57301=CARTESIAN_POINT ( 'NONE',  ( -110.4683760289727132, -287.2662352645559167, -253.7030783399848985 ) ) ;
#57302=CARTESIAN_POINT ( 'NONE',  ( -38.85363861546067454, -291.0712801540556711, -345.3458810641479317 ) ) ;
#57303=CARTESIAN_POINT ( 'NONE',  ( -55.71539521935919481, -289.8161491601089779, -197.4210253949140395 ) ) ;
#57304=CARTESIAN_POINT ( 'NONE',  ( 21.60561533811403123, -294.9154703852302077, -223.9703455894943716 ) ) ;
#57305=CARTESIAN_POINT ( 'NONE',  ( -67.87156488716884439, -284.4042948232743697, -336.9293972649542752 ) ) ;
#57306=CARTESIAN_POINT ( 'NONE',  ( -35.04263018413994502, -294.0810897534220771, -195.2167780110804358 ) ) ;
#57309=CARTESIAN_POINT ( 'NONE',  ( -60.39249233915681714, -275.7347405013114781, -198.5636014117943944 ) ) ;
#57310=CARTESIAN_POINT ( 'NONE',  ( 34.09587835474437867, -280.9571334538154588, -286.1495348777308436 ) ) ;
#57311=CARTESIAN_POINT ( 'NONE',  ( -74.81765440468608119, -281.5504951712472348, -335.3860967848603991 ) ) ;
#57312=CARTESIAN_POINT ( 'NONE',  ( -112.1509457559398015, -295.5287578501248618, -287.9604542025837191 ) ) ;
#57313=CARTESIAN_POINT ( 'NONE',  ( -63.64619764083871445, -271.9443874272685093, -201.1661740105528793 ) ) ;
#57314=CARTESIAN_POINT ( 'NONE',  ( -68.66518493698950465, -275.5469084806538831, -337.9040479613337311 ) ) ;
#57315=CARTESIAN_POINT ( 'NONE',  ( -106.2741744465558469, -298.2066209120147278, -244.7278190104321425 ) ) ;
#57316=CARTESIAN_POINT ( 'NONE',  ( -49.60663242516901761, -272.4735553194852287, -194.8877169495650037 ) ) ;
#57317=CARTESIAN_POINT ( 'NONE',  ( -107.2723681662464941, -298.2810192462973191, -247.2848950909272787 ) ) ;
#57318=DIRECTION ( 'NONE',  ( -1.000000000000000000, -0.000000000000000000, -0.000000000000000000 ) ) ;
#57319=CARTESIAN_POINT ( 'NONE',  ( 1.664555189878213159, -295.3191778065638573, -332.3171145202270509 ) ) ;
#57321=CARTESIAN_POINT ( 'NONE',  ( 25.77418742970241539, -285.0196521069949540, -229.1932720331928124 ) ) ;
#57322=CARTESIAN_POINT ( 'NONE',  ( -110.3416211263863289, -272.4214311790046281, -267.6351414138766245 ) ) ;
#57323=CARTESIAN_POINT ( 'NONE',  ( -76.10672076045177903, -285.5495102620312196, -203.7694751957007213 ) ) ;
#57324=CARTESIAN_POINT ( 'NONE',  ( 18.62652873171720813, -287.9408436094007016, -323.2128128447901645 ) ) ;
#57325=CARTESIAN_POINT ( 'NONE',  ( 16.40644411584795748, -296.2735937243684816, -323.2514933945663529 ) ) ;
#57326=CARTESIAN_POINT ( 'NONE',  ( -11.60638090825217894, -290.3877722155161223, -200.0369548763536898 ) ) ;
#57327=CARTESIAN_POINT ( 'NONE',  ( -100.1111613704287890, -278.3369986359605832, -226.0423459327373337 ) ) ;
#57328=CARTESIAN_POINT ( 'NONE',  ( -54.42813229853332757, -283.3380690714490129, -195.3538533559490702 ) ) ;
#57330=CARTESIAN_POINT ( 'NONE',  ( 28.57768800970790224, -286.7819211596159334, -302.6374989932680819 ) ) ;
#57332=CARTESIAN_POINT ( 'NONE',  ( 15.47422765890346419, -286.3052212953550679, -323.6103284888396274 ) ) ;
#57333=CARTESIAN_POINT ( 'NONE',  ( -109.2611973564170711, -298.3682866332154617, -253.8073771302953219 ) ) ;
#57334=CARTESIAN_POINT ( 'NONE',  ( -1.428545143471469103, -281.9441730135347370, -202.9159432622016936 ) ) ;
#57335=CARTESIAN_POINT ( 'NONE',  ( -98.57007099884434353, -295.1670924467572945, -226.4351187910079659 ) ) ;
#57336=CARTESIAN_POINT ( 'NONE',  ( 31.07030355454676496, -281.2106873776272664, -244.7445871767365304 ) ) ;
#57337=CARTESIAN_POINT ( 'NONE',  ( -86.39368527885039839, -295.8784943767423670, -329.7151638198332648 ) ) ;
#57338=CARTESIAN_POINT ( 'NONE',  ( -90.55984317352236701, -298.8016330983899138, -219.3122210049654939 ) ) ;
#57339=CARTESIAN_POINT ( 'NONE',  ( -15.80013513929826807, -284.4083932734251903, -197.8824834857215080 ) ) ;
#57341=CARTESIAN_POINT ( 'NONE',  ( -34.02975750886035655, -282.0939795243029380, -195.4342757497672380 ) ) ;
#57343=CARTESIAN_POINT ( 'NONE',  ( -82.07840579873577269, -296.4840181938811838, -212.3137906870738050 ) ) ;
#57345=DIRECTION ( 'NONE',  ( 0.000000000000000000, 0.000000000000000000, 1.000000000000000000 ) ) ;
#57346=CARTESIAN_POINT ( 'NONE',  ( 8.830721140459937502, -284.3957791549856324, -329.0782714599445740 ) ) ;
#57348=CARTESIAN_POINT ( 'NONE',  ( -20.19161114001082069, -289.7666405000204009, -195.3683826091709363 ) ) ;
#57349=CARTESIAN_POINT ( 'NONE',  ( 35.57996422771566358, -274.4419066435889363, -245.9737148925808583 ) ) ;
#57350=CARTESIAN_POINT ( 'NONE',  ( -37.54781906493271038, -291.8828564907146870, -197.3489651963502922 ) ) ;
#57351=CARTESIAN_POINT ( 'NONE',  ( 31.71327903191885511, -282.7305645020238103, -244.4831765541178754 ) ) ;
#57352=CARTESIAN_POINT ( 'NONE',  ( 17.13530689902991355, -277.8588632816119457, -320.1664778849046229 ) ) ;
#57353=CARTESIAN_POINT ( 'NONE',  ( 20.84004401143931773, -279.7205639435949820, -225.5968010284620107 ) ) ;
#57354=CARTESIAN_POINT ( 'NONE',  ( -109.0207153024304461, -280.2657354849513922, -292.6056084190050797 ) ) ;
#57355=CARTESIAN_POINT ( 'NONE',  ( -93.17362774639011036, -273.4436849761018493, -217.3155065374579067 ) ) ;
#57356=CARTESIAN_POINT ( 'NONE',  ( 36.06199122632855847, -275.6777916550140617, -293.6183340681683944 ) ) ;
#57357=CARTESIAN_POINT ( 'NONE',  ( 15.88844557785086486, -294.7332305639542938, -218.2501570742107617 ) ) ;
#57361=CARTESIAN_POINT ( 'NONE',  ( -32.12164970490687210, -293.1265817275605627, -345.9589239379730543 ) ) ;
#57362=CARTESIAN_POINT ( 'NONE',  ( -93.82195822494607285, -272.7159802506369601, -223.9953725165841831 ) ) ;
#57363=CARTESIAN_POINT ( 'NONE',  ( 20.85156528479959093, -295.7436086463525839, -319.7195176224915940 ) ) ;
#57364=CARTESIAN_POINT ( 'NONE',  ( 13.00589969489902309, -293.9424137320066848, -212.6278701126462067 ) ) ;
#57365=CARTESIAN_POINT ( 'NONE',  ( -39.99812008847871425, -291.0856444114978103, -345.1981128541739281 ) ) ;
#57366=CARTESIAN_POINT ( 'NONE',  ( -104.7943026507509217, -276.1229172564733858, -302.8875052824417367 ) ) ;
#57367=CARTESIAN_POINT ( 'NONE',  ( -48.80594869230788646, -279.1193064502305106, -343.9654400944965005 ) ) ;
#57368=CARTESIAN_POINT ( 'NONE',  ( 4.608112535590461967, -292.5608457392605715, -331.8552430129307140 ) ) ;
#57369=CARTESIAN_POINT ( 'NONE',  ( 33.16609357196668384, -283.0536411182113170, -242.4879742690613682 ) ) ;
#57370=CARTESIAN_POINT ( 'NONE',  ( -44.03898481386116259, -284.8858097898379356, -197.3585669899016182 ) ) ;
#57372=CARTESIAN_POINT ( 'NONE',  ( -18.73434406958133280, -282.4727102347819141, -341.0241147205268248 ) ) ;
#57373=CARTESIAN_POINT ( 'NONE',  ( -11.62600901684352905, -281.4588816592911371, -198.0544428660961671 ) ) ;
#57374=CARTESIAN_POINT ( 'NONE',  ( -108.9373471170901126, -282.9988075171709738, -297.7500061991559619 ) ) ;
#57375=CARTESIAN_POINT ( 'NONE',  ( -100.0636743314286576, -280.0808015610927555, -226.1030772980930408 ) ) ;
#57376=EDGE_CURVE ( 'NONE', #51665, #60383, #62388, .T. ) ;
#57378=CARTESIAN_POINT ( 'NONE',  ( -41.32868539329093949, -278.6215798546141968, -346.5766469139779815 ) ) ;
#57379=CARTESIAN_POINT ( 'NONE',  ( 30.89617123739170168, -295.8376638359844719, -254.7536222014695397 ) ) ;
#57381=CARTESIAN_POINT ( 'NONE',  ( -35.09767873350384804, -300.0803994080620214, -195.3603442078617718 ) ) ;
#57382=CARTESIAN_POINT ( 'NONE',  ( -95.19980865361736733, -277.2251811477385672, -223.1987804174864038 ) ) ;
#57383=CARTESIAN_POINT ( 'NONE',  ( -108.5324448336631065, -292.6544777227440477, -243.6431769258493318 ) ) ;
#57384=CARTESIAN_POINT ( 'NONE',  ( 35.63700618335886361, -292.8342948545750346, -265.3175621264012420 ) ) ;
#57385=CARTESIAN_POINT ( 'NONE',  ( -99.82395989759892529, -289.4640339718997097, -315.2779471792813979 ) ) ;
#57387=CARTESIAN_POINT ( 'NONE',  ( -37.70453738457554493, -293.6313106962790584, -346.7840079776721609 ) ) ;
#57388=CARTESIAN_POINT ( 'NONE',  ( -77.46712280369970927, -283.9042138801509623, -208.3618886819575096 ) ) ;
#57389=CARTESIAN_POINT ( 'NONE',  ( -65.82239643851400501, -293.5360195313533609, -201.7929024901108619 ) ) ;
#57390=CARTESIAN_POINT ( 'NONE',  ( -2.178076673436025956, -283.8915884332506607, -334.9104808423783197 ) ) ;
#57391=CARTESIAN_POINT ( 'NONE',  ( -91.42422615991752366, -290.7400045099170143, -324.9143235846171365 ) ) ;
#57392=CARTESIAN_POINT ( 'NONE',  ( 35.74878500729256103, -282.0209714190897898, -268.5758222161654771 ) ) ;
#57393=CARTESIAN_POINT ( 'NONE',  ( 6.374744017833825716, -293.2680984406547964, -333.3294880083132057 ) ) ;
#57394=CARTESIAN_POINT ( 'NONE',  ( -5.683665189520316297, -289.4491361807248495, -340.3748855208001487 ) ) ;
#57395=CARTESIAN_POINT ( 'NONE',  ( -23.31699491914343980, -289.3699213476267005, -346.0646086733685252 ) ) ;
#57396=CARTESIAN_POINT ( 'NONE',  ( -65.09518673239152520, -285.8459649828753300, -202.7888379612027450 ) ) ;
#57397=EDGE_LOOP ( 'NONE', ( #6350, #7139 ) ) ;
#57399=CARTESIAN_POINT ( 'NONE',  ( 36.26572443762263731, -295.6413991660483589, -288.3668686721293852 ) ) ;
#57400=CARTESIAN_POINT ( 'NONE',  ( -113.4543212214506269, -295.1393464300450660, -278.1178687398328861 ) ) ;
#57401=EDGE_CURVE ( 'NONE', #78639, #10505, #81308, .T. ) ;
#57402=CARTESIAN_POINT ( 'NONE',  ( -110.3925027004790707, -277.6792061617019840, -265.1660538705651220 ) ) ;
#57403=CARTESIAN_POINT ( 'NONE',  ( -44.03115407242199808, -273.4775149411224788, -193.6607513434001930 ) ) ;
#57405=CARTESIAN_POINT ( 'NONE',  ( -76.03845361813569070, -294.0587708068583765, -333.1363986272138504 ) ) ;
#57406=CARTESIAN_POINT ( 'NONE',  ( 18.02894103180391383, -276.6193777428455860, -221.1724151326511674 ) ) ;
#57407=CARTESIAN_POINT ( 'NONE',  ( -65.00748298105752099, -271.8264483383052266, -201.4600407906339967 ) ) ;
#57408=CARTESIAN_POINT ( 'NONE',  ( 27.51609864581672582, -295.2240421961290053, -304.8295736465178720 ) ) ;
#57409=CARTESIAN_POINT ( 'NONE',  ( -73.44270288355812681, -296.6228820809637909, -334.1650651487171331 ) ) ;
#57411=CARTESIAN_POINT ( 'NONE',  ( -102.2534306852048331, -295.0584019366953612, -232.3574701437980536 ) ) ;
#57413=CARTESIAN_POINT ( 'NONE',  ( -20.54592245100773340, -298.9086733388634229, -193.4612474181249411 ) ) ;
#57414=CARTESIAN_POINT ( 'NONE',  ( -48.16543679440111703, -287.7671422057633208, -343.2014370238063066 ) ) ;
#57416=CARTESIAN_POINT ( 'NONE',  ( -104.2578474141468945, -291.0925637964194834, -300.2459760156460788 ) ) ;
#57417=CARTESIAN_POINT ( 'NONE',  ( -35.53152440351444596, -274.5666084124854365, -193.4308338995453198 ) ) ;
#57418=CARTESIAN_POINT ( 'NONE',  ( -66.83176999049480571, -297.9880627709171677, -203.5460620145148312 ) ) ;
#57419=CARTESIAN_POINT ( 'NONE',  ( -89.92879280924441332, -281.2943949284703535, -216.3160927189553320 ) ) ;
#57420=CARTESIAN_POINT ( 'NONE',  ( 39.12637323140874201, -280.2676361926265258, -272.7966935117529488 ) ) ;
#57421=CARTESIAN_POINT ( 'NONE',  ( -58.46672194941214684, -282.6667452458896719, -344.3560215239326681 ) ) ;
#57422=CARTESIAN_POINT ( 'NONE',  ( 38.12032187001884864, -274.7155055850394660, -255.5693627494779321 ) ) ;
#57423=CARTESIAN_POINT ( 'NONE',  ( 10.33847168575941211, -279.0971034108006279, -210.8540775407469994 ) ) ;
#57424=CARTESIAN_POINT ( 'NONE',  ( -8.223105111685928392, -278.4323822904095778, -201.0497082722438620 ) ) ;
#57425=CARTESIAN_POINT ( 'NONE',  ( -35.11229096291037877, -296.7654577688189192, -196.8684749249626691 ) ) ;
#57426=CARTESIAN_POINT ( 'NONE',  ( 5.250447008766406576, -276.6280386095629069, -208.5661857936225942 ) ) ;
#57428=CARTESIAN_POINT ( 'NONE',  ( 29.45292089579642436, -291.1111051836316506, -235.3648305719601979 ) ) ;
#57429=CARTESIAN_POINT ( 'NONE',  ( -25.02144037237970764, -292.2051316212854886, -194.3531499821454815 ) ) ;
#57430=CARTESIAN_POINT ( 'NONE',  ( 33.48234783454029184, -277.8796050543564320, -295.6936990262208269 ) ) ;
#57431=CARTESIAN_POINT ( 'NONE',  ( 54.50831346207038308, -297.2042866843169691, -195.5591849551906591 ) ) ;
#57432=CARTESIAN_POINT ( 'NONE',  ( -95.68723369552144220, -284.4261031900746275, -220.2817513086118595 ) ) ;
#57434=CARTESIAN_POINT ( 'NONE',  ( -90.81678182791006293, -283.2938892299598592, -217.7009102401183895 ) ) ;
#57436=CARTESIAN_POINT ( 'NONE',  ( 35.30292389297547118, -292.2095341346421264, -259.8783175064681359 ) ) ;
#57437=CARTESIAN_POINT ( 'NONE',  ( -39.99473230775556232, -284.1580448918737147, -196.1733366253405393 ) ) ;
#57440=CARTESIAN_POINT ( 'NONE',  ( -15.02125698019107070, -292.7630281929911575, -342.0174050159408239 ) ) ;
#57441=CARTESIAN_POINT ( 'NONE',  ( -92.93975391155041166, -282.3120710611309505, -322.6446473009380043 ) ) ;
#57442=CARTESIAN_POINT ( 'NONE',  ( -104.1021455952084835, -280.5741129216386298, -238.7848775330509454 ) ) ;
#57443=CARTESIAN_POINT ( 'NONE',  ( -85.27644517237906996, -286.6115746906446020, -210.6093905180191257 ) ) ;
#57444=CARTESIAN_POINT ( 'NONE',  ( -6.619247236738801554, -278.6898606552815068, -200.8480751687957309 ) ) ;
#57445=CARTESIAN_POINT ( 'NONE',  ( 35.12421513372721193, -287.6684268581126389, -279.1753749148476231 ) ) ;
#57446=CARTESIAN_POINT ( 'NONE',  ( -39.15422912802713284, -278.5006164769621932, -343.9280239747898236 ) ) ;
#57447=CARTESIAN_POINT ( 'NONE',  ( -94.92427309393181645, -279.9900994756662271, -225.2094862833691877 ) ) ;
#57448=CARTESIAN_POINT ( 'NONE',  ( 6.564666552719763182, -288.6251064464843807, -209.0544150087766297 ) ) ;
#57450=CARTESIAN_POINT ( 'NONE',  ( -14.80798891540781703, -298.1603007223051804, -193.3617316766313365 ) ) ;
#57451=CARTESIAN_POINT ( 'NONE',  ( -34.49047466810819174, -290.9961725953706377, -345.0021454943353092 ) ) ;
#57452=CARTESIAN_POINT ( 'NONE',  ( 114.7448031289451222, -299.5541904835127980, -195.3611179825600175 ) ) ;
#57453=CARTESIAN_POINT ( 'NONE',  ( 36.60358173371528068, -284.4805209788416391, -305.9350535429201159 ) ) ;
#57455=CARTESIAN_POINT ( 'NONE',  ( -52.15869887680651829, -271.8628675873937937, -196.6161525834573069 ) ) ;
#57456=CARTESIAN_POINT ( 'NONE',  ( 12.85337300930843796, -292.7655053564891432, -327.7625101204392308 ) ) ;
#57457=CARTESIAN_POINT ( 'NONE',  ( 20.87660219277669071, -288.4418524621688675, -225.1799600806849071 ) ) ;
#57458=CARTESIAN_POINT ( 'NONE',  ( 35.32491623878451037, -283.1285609269580732, -256.2396718144761962 ) ) ;
#57459=CARTESIAN_POINT ( 'NONE',  ( -3.306755722038154932, -290.0368838014886137, -338.7878341351317886 ) ) ;
#57460=CARTESIAN_POINT ( 'NONE',  ( 19.27068535932135518, -289.5713675161308061, -321.8426233913722854 ) ) ;
#57461=CARTESIAN_POINT ( 'NONE',  ( -38.90182529045613080, -285.0718496041399703, -345.3577273792831761 ) ) ;
#57462=CARTESIAN_POINT ( 'NONE',  ( -77.81309571363084387, -277.7461388081583777, -335.9293076122339698 ) ) ;
#57464=CARTESIAN_POINT ( 'NONE',  ( 35.69820681772038995, -291.8788896556168311, -289.7127637497367800 ) ) ;
#57465=CARTESIAN_POINT ( 'NONE',  ( 34.58674983517818191, -281.7334086162607036, -297.8438050850731429 ) ) ;
#57466=CARTESIAN_POINT ( 'NONE',  ( -110.8086392094458148, -274.5553242645343062, -259.3566200948133087 ) ) ;
#57467=CARTESIAN_POINT ( 'NONE',  ( -20.19161114001083490, -297.3376638359846424, -345.3538533559490702 ) ) ;
#57469=CARTESIAN_POINT ( 'NONE',  ( 33.78127118843386256, -273.4491020623128179, -243.6123429966363290 ) ) ;
#57471=CARTESIAN_POINT ( 'NONE',  ( -38.34840713683026081, -279.5468517500289636, -197.2941042146621555 ) ) ;
#57472=CARTESIAN_POINT ( 'NONE',  ( 38.92044695501905238, -276.6597244229483294, -262.6052091167042590 ) ) ;
#57474=CARTESIAN_POINT ( 'NONE',  ( -67.07391652680202299, -299.0798773384724427, -203.0318728111311657 ) ) ;
#57475=CARTESIAN_POINT ( 'NONE',  ( -102.7239680373683939, -283.0835743896361123, -310.5852308455691855 ) ) ;
#57476=CARTESIAN_POINT ( 'NONE',  ( -97.59924262571209397, -292.9055114984050761, -227.2976267820473311 ) ) ;
#57477=CARTESIAN_POINT ( 'NONE',  ( -8.017483454247686936, -276.0299203628094347, -199.9735394664015473 ) ) ;
#57478=CARTESIAN_POINT ( 'NONE',  ( 75.64300948861529150, -300.6422523422198765, -193.7355811110692514 ) ) ;
#57479=CARTESIAN_POINT ( 'NONE',  ( 0.1828843131839977265, -296.5518716174549354, -335.1654164980282076 ) ) ;
#57480=CARTESIAN_POINT ( 'NONE',  ( -21.01236473298763840, -280.8421099590888730, -343.4444356548648329 ) ) ;
#57481=CARTESIAN_POINT ( 'NONE',  ( -104.5894439127878286, -290.7046806034951487, -232.8979994883202096 ) ) ;
#57482=CARTESIAN_POINT ( 'NONE',  ( 28.19914733018943309, -274.0504545713945959, -306.1936657736611664 ) ) ;
#57483=CARTESIAN_POINT ( 'NONE',  ( 21.45970611976892428, -288.4942443646540937, -221.8963365288080070 ) ) ;
#57484=CARTESIAN_POINT ( 'NONE',  ( -55.07387260789974448, -290.7390208761353847, -199.2288740154367304 ) ) ;
#57486=CARTESIAN_POINT ( 'NONE',  ( -102.7023446523637062, -289.6486321728741586, -230.6789404729901491 ) ) ;
#57487=CARTESIAN_POINT ( 'NONE',  ( -94.96987217696947425, -289.5870084009867469, -315.2264019682011735 ) ) ;
#57489=CARTESIAN_POINT ( 'NONE',  ( -33.75559207112330995, -287.1759547169260145, -193.7541186985337163 ) ) ;
#57490=CARTESIAN_POINT ( 'NONE',  ( -70.45859756778790484, -277.8346326625081701, -335.4407506707237872 ) ) ;
#57491=CARTESIAN_POINT ( 'NONE',  ( 38.29911383466275510, -292.6322949907391830, -283.0881241972736007 ) ) ;
#57492=CARTESIAN_POINT ( 'NONE',  ( -69.13672567637179611, -284.1108815746687242, -340.3925753331854480 ) ) ;
#57493=CARTESIAN_POINT ( 'NONE',  ( -68.49609166267092064, -285.9871739795202643, -199.9539318047604581 ) ) ;
#57494=CARTESIAN_POINT ( 'NONE',  ( -39.70616826000728850, -280.3549584877739562, -197.3657419946568155 ) ) ;
#57495=CARTESIAN_POINT ( 'NONE',  ( 189.8312124288175085, 271.3805950635771751, -139.6404239813599304 ) ) ;
#57496=CARTESIAN_POINT ( 'NONE',  ( -40.70455346190973955, -139.0725253683308722, -363.9141075947721902 ) ) ;
#57497=CARTESIAN_POINT ( 'NONE',  ( -112.4672374317974288, -270.5562577345839941, -270.3357054654630360 ) ) ;
#57498=CARTESIAN_POINT ( 'NONE',  ( -110.3491504304166284, -271.8213126082049484, -264.8912199137930088 ) ) ;
#57499=CARTESIAN_POINT ( 'NONE',  ( 13.72178132048049548, -273.7089601221063617, -217.7612421696789795 ) ) ;
#57500=CARTESIAN_POINT ( 'NONE',  ( -77.05584084700134895, -295.0765672385900302, -336.3193379948940560 ) ) ;
#57501=CARTESIAN_POINT ( 'NONE',  ( 203.3291423003342402, 291.9839310567934376, -68.27044577648942436 ) ) ;
#57502=CARTESIAN_POINT ( 'NONE',  ( -78.56167357764061876, -272.1943012040609915, -205.9079407074285086 ) ) ;
#57503=CARTESIAN_POINT ( 'NONE',  ( -67.33984280108882103, -299.5149506334882972, -202.4430297835519923 ) ) ;
#57504=CARTESIAN_POINT ( 'NONE',  ( -13.10958062581066663, -290.0457929119829714, -339.7444579282480390 ) ) ;
#57505=CARTESIAN_POINT ( 'NONE',  ( -32.14905656049183591, -293.1988296695339500, -197.2234654142295653 ) ) ;
#57507=CARTESIAN_POINT ( 'NONE',  ( -113.1590559064126182, -297.6452695913094431, -258.2549207732910190 ) ) ;
#57508=CARTESIAN_POINT ( 'NONE',  ( -68.80711504432673564, -286.1193169480072243, -204.4085862466549202 ) ) ;
#57509=CARTESIAN_POINT ( 'NONE',  ( -19.31522148232867409, -295.6289003107107192, -345.1099654740436904 ) ) ;
#57510=CARTESIAN_POINT ( 'NONE',  ( -19.29562548196082261, -295.3184648878237226, -345.2081133636395975 ) ) ;
#57511=CARTESIAN_POINT ( 'NONE',  ( -7.272185374082278386, -292.6245777682630660, -203.8417652572911436 ) ) ;
#57513=CARTESIAN_POINT ( 'NONE',  ( -73.28189792807118863, -275.4999379333262937, -203.8377942409727552 ) ) ;
#57516=CARTESIAN_POINT ( 'NONE',  ( -108.4533884341641681, -278.4334072384455681, -240.9901341833195829 ) ) ;
#57517=CARTESIAN_POINT ( 'NONE',  ( -32.61971085465124531, -272.5124925270429230, -196.6996715409798071 ) ) ;
#57518=CARTESIAN_POINT ( 'NONE',  ( -35.82054257266347719, -299.2766886233366677, -196.9637219586092272 ) ) ;
#57519=CARTESIAN_POINT ( 'NONE',  ( 34.06049168239887592, -276.2786328182733655, -254.0221106799102131 ) ) ;
#57520=CARTESIAN_POINT ( 'NONE',  ( -60.58279208308476882, -275.5150249246643739, -197.9610297328918023 ) ) ;
#57521=CARTESIAN_POINT ( 'NONE',  ( 35.69734559211168090, -273.3352183382182830, -251.8218459788683674 ) ) ;
#57522=CARTESIAN_POINT ( 'NONE',  ( -90.47562891886720138, -296.4807032040559989, -320.6403648810660911 ) ) ;
#57523=CARTESIAN_POINT ( 'NONE',  ( 36.23026466787008104, -292.1683708186756121, -273.5323196196504227 ) ) ;
#57525=CARTESIAN_POINT ( 'NONE',  ( -98.53123169608137744, -279.6669738137275658, -223.6988127938673188 ) ) ;
#57526=CARTESIAN_POINT ( 'NONE',  ( -19.01489548267566931, -276.9762709553095874, -341.0231886851154286 ) ) ;
#57527=CARTESIAN_POINT ( 'NONE',  ( 33.40980844623978641, -285.8630855169132019, -241.1104052066764325 ) ) ;
#57528=CARTESIAN_POINT ( 'NONE',  ( -95.08626478697190976, -297.8890205379088911, -318.5017388261641713 ) ) ;
#57529=CARTESIAN_POINT ( 'NONE',  ( 82.67955185657098127, -297.1469379644294690, -196.0571845609111676 ) ) ;
#57530=CARTESIAN_POINT ( 'NONE',  ( 1.388417528942380130, -287.7172745274576187, -332.4302706520730339 ) ) ;
#57531=CARTESIAN_POINT ( 'NONE',  ( -101.6818008781638270, -277.2862049186804825, -233.7779873481170796 ) ) ;
#57532=CARTESIAN_POINT ( 'NONE',  ( -105.8227089317481102, -276.7695067987242510, -297.3004266075571422 ) ) ;
#57534=CARTESIAN_POINT ( 'NONE',  ( -91.20241366768098601, -285.8174500044536330, -322.6261013126309649 ) ) ;
#57535=CARTESIAN_POINT ( 'NONE',  ( -1.261726975119667138, -277.7676061218281802, -334.3355042765239205 ) ) ;
#57537=CARTESIAN_POINT ( 'NONE',  ( 15.48722516338289701, -273.1841680084531845, -215.4471391912374827 ) ) ;
#57539=CARTESIAN_POINT ( 'NONE',  ( -14.04079314414769541, -275.0139992882502042, -201.0721549237471493 ) ) ;
#57540=CARTESIAN_POINT ( 'NONE',  ( 19.65880231802498557, -282.8745502591153809, -221.3418491594536022 ) ) ;
#57542=CARTESIAN_POINT ( 'NONE',  ( 37.91799713514392067, -289.3794014643193009, -263.0714025925938699 ) ) ;
#57543=CARTESIAN_POINT ( 'NONE',  ( 34.12147472795849978, -291.8476754347890392, -293.2889027800566168 ) ) ;
#57544=CARTESIAN_POINT ( 'NONE',  ( -3.044879762945660762, -290.6499362809184390, -204.5234874394981830 ) ) ;
#57545=CARTESIAN_POINT ( 'NONE',  ( 197.0349383350915105, 285.8449894349855640, -111.9383547020201064 ) ) ;
#57547=CARTESIAN_POINT ( 'NONE',  ( -29.07173506878448421, -287.4291689893769899, -346.2713652077850384 ) ) ;
#57548=CARTESIAN_POINT ( 'NONE',  ( -113.3421064416752415, -282.7611768888026518, -272.7941257223787375 ) ) ;
#57549=CARTESIAN_POINT ( 'NONE',  ( 10.30390055809582073, -283.8052355891049388, -326.5108663641944418 ) ) ;
#57550=CARTESIAN_POINT ( 'NONE',  ( -110.2558626212838249, -285.2758752858072171, -276.3716615982054918 ) ) ;
#57551=CARTESIAN_POINT ( 'NONE',  ( -39.19702060236851793, -294.0088967395003579, -195.0160007210211006 ) ) ;
#57552=CARTESIAN_POINT ( 'NONE',  ( -96.01432809815464964, -273.5575610569894707, -220.5084318510457706 ) ) ;
#57553=CARTESIAN_POINT ( 'NONE',  ( -94.38751466024767467, -287.9495505450739756, -319.9099751280563737 ) ) ;
#57554=CARTESIAN_POINT ( 'NONE',  ( -11.86618473281223984, -276.7296215459751352, -343.0806402270740136 ) ) ;
#57555=CARTESIAN_POINT ( 'NONE',  ( 35.55064936178566626, -295.3238391607541757, -254.2225455095673965 ) ) ;
#57557=CARTESIAN_POINT ( 'NONE',  ( 21.27581636871892101, -295.4090924074130839, -223.5744983911110353 ) ) ;
#57558=CARTESIAN_POINT ( 'NONE',  ( -96.15056012248865613, -283.8515532328726181, -226.2843501182847490 ) ) ;
#57560=CARTESIAN_POINT ( 'NONE',  ( -93.44824617194852578, -277.2443382491358079, -220.5910854179329021 ) ) ;
#57562=CARTESIAN_POINT ( 'NONE',  ( -23.51977760728848565, -296.6223423666537542, -194.1648020273771920 ) ) ;
#57563=CARTESIAN_POINT ( 'NONE',  ( 35.48054327527929530, -274.8092888467007811, -263.4193056203586139 ) ) ;
#57564=CARTESIAN_POINT ( 'NONE',  ( 31.46893760137199791, -294.7232905918149299, -243.9830231589062919 ) ) ;
#57565=CARTESIAN_POINT ( 'NONE',  ( 15.03543220320434060, -293.7544863068172276, -219.1021266316067511 ) ) ;
#57566=CARTESIAN_POINT ( 'NONE',  ( -110.7375220870011674, -297.5941631761612598, -292.0024666298239708 ) ) ;
#57567=CARTESIAN_POINT ( 'NONE',  ( -108.5923327975898189, -296.1759162869379907, -286.2465625383132988 ) ) ;
#57568=CARTESIAN_POINT ( 'NONE',  ( -107.9058994637561426, -292.2229007728791998, -295.7716358734990081 ) ) ;
#57569=CARTESIAN_POINT ( 'NONE',  ( -58.48471078639734344, -283.4847068076434198, -344.4569637422487176 ) ) ;
#57570=CARTESIAN_POINT ( 'NONE',  ( -34.13143451227233527, -272.2317130023740219, -194.6643566445341378 ) ) ;
#57571=CARTESIAN_POINT ( 'NONE',  ( -12.70170037734914459, -286.1971713319660466, -197.4099670884224338 ) ) ;
#57572=CARTESIAN_POINT ( 'NONE',  ( -109.7618603081762956, -280.2979932529585767, -288.5015011253096873 ) ) ;
#57573=CARTESIAN_POINT ( 'NONE',  ( -99.80375660342556898, -284.1372199172582214, -232.0297216355389196 ) ) ;
#57574=CARTESIAN_POINT ( 'NONE',  ( -67.27956021383455720, -287.4445661254218862, -339.1268448000188300 ) ) ;
#57575=CARTESIAN_POINT ( 'NONE',  ( 0.9968329295543288948, -56.25428601379442028, -352.6033083298257225 ) ) ;
#57576=CARTESIAN_POINT ( 'NONE',  ( 33.09025846622809297, -286.8033436812949049, -250.9361945500980937 ) ) ;
#57577=CARTESIAN_POINT ( 'NONE',  ( 31.65710497515726018, -282.3267508583586505, -236.9649168505702050 ) ) ;
#57578=CARTESIAN_POINT ( 'NONE',  ( -38.92736724058741515, -288.1303435202926266, -347.1094461313792294 ) ) ;
#57579=CARTESIAN_POINT ( 'NONE',  ( -86.30641667149771479, -280.9862158008576216, -211.9065678579501082 ) ) ;
#57580=CARTESIAN_POINT ( 'NONE',  ( -79.65209336095861659, -280.8088368804564539, -206.5548815688834736 ) ) ;
#57581=CARTESIAN_POINT ( 'NONE',  ( -100.8107603293378105, -278.8794095190371536, -234.2961987166378037 ) ) ;
#57582=CARTESIAN_POINT ( 'NONE',  ( -65.20566783748141404, -275.6661365040711758, -201.0981725180516548 ) ) ;
#57583=CARTESIAN_POINT ( 'NONE',  ( 38.85189671985328630, -293.4086737227804633, -258.8886978729627231 ) ) ;
#57584=CARTESIAN_POINT ( 'NONE',  ( 24.86663278337135097, -286.1324089665666293, -311.6393937252423143 ) ) ;
#57585=CARTESIAN_POINT ( 'NONE',  ( -7.522245727649240266, -294.0367257180901674, -200.2239083111984712 ) ) ;
#57586=CARTESIAN_POINT ( 'NONE',  ( -92.06652339558283415, -296.1670981600845494, -221.5818212222534953 ) ) ;
#57587=CARTESIAN_POINT ( 'NONE',  ( -61.98888978234186453, -285.2950950539051291, -340.6566255807605330 ) ) ;
#57588=CARTESIAN_POINT ( 'NONE',  ( -103.9576467496765844, -295.8146593540945446, -300.3913091889525617 ) ) ;
#57589=CARTESIAN_POINT ( 'NONE',  ( 3.963421869051978685, -293.6738002830130654, -205.6810023701736156 ) ) ;
#57590=CARTESIAN_POINT ( 'NONE',  ( -19.51771992270131761, -280.9387964671371378, -199.4130698934563952 ) ) ;
#57591=CARTESIAN_POINT ( 'NONE',  ( 35.51047184528718503, -274.3035095503947787, -245.9988246046506504 ) ) ;
#57592=CARTESIAN_POINT ( 'NONE',  ( -102.2108058144700209, -290.6604256641449524, -311.7545139252495687 ) ) ;
#57593=CARTESIAN_POINT ( 'NONE',  ( -31.75145080200277192, -281.1219192954770847, -345.9324591248744696 ) ) ;
#57594=CARTESIAN_POINT ( 'NONE',  ( -106.4926509162334014, -290.4496337232558290, -304.3037160059258781 ) ) ;
#57595=CARTESIAN_POINT ( 'NONE',  ( 34.01576570316509418, -287.6810441981606346, -254.8627452610713249 ) ) ;
#57597=CARTESIAN_POINT ( 'NONE',  ( 63.26945853893380445, 48.02268529798013219, -317.1124933380390871 ) ) ;
#57598=CARTESIAN_POINT ( 'NONE',  ( 188.3815699774405914, 268.4127512313500006, -137.5006950848226097 ) ) ;
#57600=CARTESIAN_POINT ( 'NONE',  ( -107.9788296581491238, -277.4982106727002247, -289.4136154328065231 ) ) ;
#57601=EDGE_LOOP ( 'NONE', ( #65563, #58869 ) ) ;
#57602=CARTESIAN_POINT ( 'NONE',  ( -5.411485193063779064, -279.4027938030335463, -204.3710623003073579 ) ) ;
#57603=CARTESIAN_POINT ( 'NONE',  ( -15.77921187233445188, -273.9902756953135849, -196.4085443027745441 ) ) ;
#57604=CARTESIAN_POINT ( 'NONE',  ( 162.4344822024288248, 217.7039127420125055, -203.2254006442507546 ) ) ;
#57605=CARTESIAN_POINT ( 'NONE',  ( -90.63410881575923383, -277.8897790276416799, -215.5285787958924288 ) ) ;
#57606=CARTESIAN_POINT ( 'NONE',  ( -43.08405447717554182, -281.1449700493054138, -344.8359323433271584 ) ) ;
#57607=CARTESIAN_POINT ( 'NONE',  ( -99.11106645259468451, -298.9065216928514133, -226.1059555853186112 ) ) ;
#57608=CARTESIAN_POINT ( 'NONE',  ( -92.60715282538144777, -291.7248562719928486, -222.5728539424964367 ) ) ;
#57609=CARTESIAN_POINT ( 'NONE',  ( 19.88702626850750121, -286.8845445538771060, -316.4709472460172606 ) ) ;
#57610=CARTESIAN_POINT ( 'NONE',  ( 29.85441887773816205, -275.7170070474711565, -232.8618800972456313 ) ) ;
#57611=CARTESIAN_POINT ( 'NONE',  ( -81.07100676322005484, -273.4395754160483420, -211.8447354645772975 ) ) ;
#57612=ORIENTED_EDGE ( 'NONE', *, *, #59748, .T. ) ;
#57614=DIRECTION ( 'NONE',  ( 0.000000000000000000, 0.000000000000000000, -1.000000000000000000 ) ) ;
#57615=CARTESIAN_POINT ( 'NONE',  ( -96.58341530287106025, -281.1118303149219173, -223.4598025867872195 ) ) ;
#57617=CARTESIAN_POINT ( 'NONE',  ( -4.220160341655663672, -281.5790929561746907, -204.9469422431492092 ) ) ;
#57618=CARTESIAN_POINT ( 'NONE',  ( -73.30608116431800170, -281.3421103969245110, -203.4095462067143103 ) ) ;
#57619=CARTESIAN_POINT ( 'NONE',  ( -85.02402419621715524, -282.7882321303009689, -325.9471271835198536 ) ) ;
#57620=CARTESIAN_POINT ( 'NONE',  ( -108.2902308738619865, -280.1260134859790583, -292.3773211751072267 ) ) ;
#57621=CARTESIAN_POINT ( 'NONE',  ( -33.98995736025342751, -272.5749491994733376, -196.7440440525120664 ) ) ;
#57624=CARTESIAN_POINT ( 'NONE',  ( -5.342680378161870358, -277.4445369737171632, -340.2197005346345122 ) ) ;
#57626=CARTESIAN_POINT ( 'NONE',  ( -77.52063042724746822, -276.1544430970827761, -335.4169187851539391 ) ) ;
#57629=CARTESIAN_POINT ( 'NONE',  ( -65.92841814486052954, -285.4041819847944907, -340.0973504368578801 ) ) ;
#57630=CARTESIAN_POINT ( 'NONE',  ( 20.64494854287097425, -293.3760144242928618, -314.9927269770820430 ) ) ;
#57631=CARTESIAN_POINT ( 'NONE',  ( 38.57299032387706461, -287.0583064800667330, -282.9432084051824177 ) ) ;
#57632=CARTESIAN_POINT ( 'NONE',  ( -71.62801043384467903, -283.8324818411110755, -204.7682605885046314 ) ) ;
#57633=CARTESIAN_POINT ( 'NONE',  ( -109.7697552912194112, -283.2981983729380318, -257.2691202428175075 ) ) ;
#57634=CARTESIAN_POINT ( 'NONE',  ( -0.5063166204722437946, -286.7956963449546492, -334.6161180392822416 ) ) ;
#57635=CARTESIAN_POINT ( 'NONE',  ( 35.82618576950239486, -282.8413288285244676, -276.7706258523944030 ) ) ;
#57636=CARTESIAN_POINT ( 'NONE',  ( -60.23573534587868750, -271.7553288428964606, -198.8866080079085066 ) ) ;
#57637=CARTESIAN_POINT ( 'NONE',  ( -100.7647246949549498, -282.3892267799135993, -312.6927860890463649 ) ) ;
#57638=CARTESIAN_POINT ( 'NONE',  ( -112.3383107573079798, -298.5614778680699146, -269.6476477581690574 ) ) ;
#57639=CARTESIAN_POINT ( 'NONE',  ( -3.036338252101231650, -284.5041144381829099, -203.4649488932181782 ) ) ;
#57640=CARTESIAN_POINT ( 'NONE',  ( -110.2014851540139517, -279.5972040903377547, -262.4675300087862411 ) ) ;
#57641=CARTESIAN_POINT ( 'NONE',  ( -0.6343007329302595698, -288.5387744382253459, -204.7522600594095081 ) ) ;
#57644=CARTESIAN_POINT ( 'NONE',  ( 16.44701099991650395, -294.7288609567850131, -217.2206352423231408 ) ) ;
#57645=CARTESIAN_POINT ( 'NONE',  ( -110.5536585615042071, -276.7617036329259577, -254.0232976385879340 ) ) ;
#57646=CARTESIAN_POINT ( 'NONE',  ( -105.0185882149049661, -289.2778948186726211, -306.7478963356214194 ) ) ;
#57647=CARTESIAN_POINT ( 'NONE',  ( 30.21428099867172534, -292.3473855861907964, -300.0702045916698921 ) ) ;
#57648=CARTESIAN_POINT ( 'NONE',  ( -74.74242456649125188, -278.2282962507962338, -207.0378750661772358 ) ) ;
#57649=CARTESIAN_POINT ( 'NONE',  ( -60.88556721353560164, -295.8830671455014567, -199.9039678419400445 ) ) ;
#57650=CARTESIAN_POINT ( 'NONE',  ( -94.68615157272625993, -292.5127691080730870, -224.3752867370811828 ) ) ;
#57651=CARTESIAN_POINT ( 'NONE',  ( 39.58706461736020543, -278.0519495502701943, -270.3284710469133074 ) ) ;
#57652=CARTESIAN_POINT ( 'NONE',  ( 0.1825307035090767416, -293.0418556664899938, -336.8189151771805996 ) ) ;
#57653=CARTESIAN_POINT ( 'NONE',  ( -5.428240273270160898, -290.2252231001308473, -336.9041228582225358 ) ) ;
#57654=CARTESIAN_POINT ( 'NONE',  ( 22.32648821661240035, -291.1541520665195435, -223.2905424537789827 ) ) ;
#57655=CARTESIAN_POINT ( 'NONE',  ( 23.24525375620302725, -289.5547145105940672, -312.1516973993332158 ) ) ;
#57657=CARTESIAN_POINT ( 'NONE',  ( -80.49452319113039778, -290.4565588084187198, -329.5040613568885419 ) ) ;
#57660=CARTESIAN_POINT ( 'NONE',  ( -54.39819252439830422, -290.4714984615385447, -345.0954274552201468 ) ) ;
#57661=CARTESIAN_POINT ( 'NONE',  ( 11.93602529117274003, -278.7532210193863307, -213.3513593664415282 ) ) ;
#57662=CARTESIAN_POINT ( 'NONE',  ( -96.76136113481905454, -291.1456545598753110, -227.8692024489122048 ) ) ;
#57663=CARTESIAN_POINT ( 'NONE',  ( -31.07971276210952638, -280.4623679564709278, -193.5847048088081124 ) ) ;
#57665=CARTESIAN_POINT ( 'NONE',  ( 36.58060354450348228, -280.9489441826681286, -248.8374167656960196 ) ) ;
#57666=CARTESIAN_POINT ( 'NONE',  ( 14.54099637844502624, -284.7815316527086793, -216.1305425700780347 ) ) ;
#57668=CARTESIAN_POINT ( 'NONE',  ( 4.059782309532352862, -280.6278472192745994, -332.0413240862674229 ) ) ;
#57670=CARTESIAN_POINT ( 'NONE',  ( -49.00783483711197164, -283.9034929596534766, -196.2216557077590551 ) ) ;
#57671=CARTESIAN_POINT ( 'NONE',  ( 202.9739431621297854, 291.9636489107636521, -68.24819746054791381 ) ) ;
#57672=CARTESIAN_POINT ( 'NONE',  ( -94.43010240320995763, -277.7242992126917898, -219.7288942586965845 ) ) ;
#57673=CARTESIAN_POINT ( 'NONE',  ( -80.75186664459556596, -284.3989256426984866, -207.0747983761724527 ) ) ;
#57674=CARTESIAN_POINT ( 'NONE',  ( -44.60430831433531296, -298.8993966867382142, -197.4362778230943150 ) ) ;
#57676=CARTESIAN_POINT ( 'NONE',  ( -109.4969901315334084, -292.3544543350430445, -254.8674243629021703 ) ) ;
#57677=CARTESIAN_POINT ( 'NONE',  ( 24.83677692059092834, -276.3843068797114597, -225.9265440971653049 ) ) ;
#57678=CARTESIAN_POINT ( 'NONE',  ( 23.99984261568192778, -275.7682446408014130, -310.0687669069876620 ) ) ;
#57679=CARTESIAN_POINT ( 'NONE',  ( 11.61579823217088325, -296.3728436956533869, -327.1780520793758456 ) ) ;
#57680=CARTESIAN_POINT ( 'NONE',  ( -54.49954988508929432, -289.4332698593926239, -345.4798568130370313 ) ) ;
#57681=CARTESIAN_POINT ( 'NONE',  ( 25.51024815650696098, -280.1945943937059269, -312.3009176333296750 ) ) ;
#57682=CARTESIAN_POINT ( 'NONE',  ( 24.81570823793426328, -292.7820934494729386, -224.9138233464549899 ) ) ;
#57683=CARTESIAN_POINT ( 'NONE',  ( -22.68185010900764098, -291.3031649485820935, -198.6080884659516528 ) ) ;
#57684=CARTESIAN_POINT ( 'NONE',  ( -80.73583205035789945, -293.6402437740788400, -331.5960433192204846 ) ) ;
#57687=CARTESIAN_POINT ( 'NONE',  ( -20.05152557198974961, -291.7879154240641810, -199.3226196073275389 ) ) ;
#57689=CARTESIAN_POINT ( 'NONE',  ( 7.399455738971487229, -273.9094976428776818, -326.5171145203363494 ) ) ;
#57690=CARTESIAN_POINT ( 'NONE',  ( -110.5789246492023636, -295.3204737289673858, -293.4079454594493654 ) ) ;
#57691=CARTESIAN_POINT ( 'NONE',  ( -70.24276363978646032, -284.7917795042565103, -339.4465961953549140 ) ) ;
#57692=CARTESIAN_POINT ( 'NONE',  ( -79.30754879394638124, -285.3015876465173051, -210.5674323561158303 ) ) ;
#57693=CARTESIAN_POINT ( 'NONE',  ( 17.96830438507194216, -277.7612621640561201, -319.0783250915033591 ) ) ;
#57694=CARTESIAN_POINT ( 'NONE',  ( 20.96305535833123912, -292.2163899682133774, -316.9905213263956512 ) ) ;
#57695=CARTESIAN_POINT ( 'NONE',  ( 34.76771298962304257, -295.5299694093850462, -287.0965520938358964 ) ) ;
#57696=CARTESIAN_POINT ( 'NONE',  ( -4.904341022967168229, -275.4101915475108058, -336.2154066289202774 ) ) ;
#57699=CARTESIAN_POINT ( 'NONE',  ( 37.07503850517524313, -293.4655059971601645, -290.0561250347504370 ) ) ;
#57700=CARTESIAN_POINT ( 'NONE',  ( 15.11513296530155337, -290.2249039928973957, -323.1777333471455904 ) ) ;
#57702=CARTESIAN_POINT ( 'NONE',  ( -97.51076072415143869, -274.3945810059534551, -222.9512786293650777 ) ) ;
#57703=CARTESIAN_POINT ( 'NONE',  ( 6.982152532026011826, -287.3249466757657160, -212.1655164235480981 ) ) ;
#57705=CARTESIAN_POINT ( 'NONE',  ( -96.62803972800544727, -278.2681686192193524, -221.5764506891514714 ) ) ;
#57706=CARTESIAN_POINT ( 'NONE',  ( 22.21296548495133649, -294.8576103732307843, -319.0290388311582319 ) ) ;
#57707=CARTESIAN_POINT ( 'NONE',  ( -26.34757877042141772, -287.0532333732097072, -345.3240072952887090 ) ) ;
#57708=CARTESIAN_POINT ( 'NONE',  ( -50.45974191532993558, -295.5484066936854788, -346.2679400626686288 ) ) ;
#57709=CARTESIAN_POINT ( 'NONE',  ( 18.49001247015401006, -293.2169807820790197, -223.2983157370485117 ) ) ;
#57713=CARTESIAN_POINT ( 'NONE',  ( -7.631111581328803517, -287.9545692886845814, -200.0199270819602191 ) ) ;
#57714=CARTESIAN_POINT ( 'NONE',  ( -2.602324593224659921, -283.9809262143061233, -198.2974183793908196 ) ) ;
#57716=CARTESIAN_POINT ( 'NONE',  ( -71.18225273169647949, -278.9657088200427779, -201.3094721902065487 ) ) ;
#57717=CARTESIAN_POINT ( 'NONE',  ( 4.434289685649758006, -284.4878019350697400, -332.5108090149890927 ) ) ;
#57718=CARTESIAN_POINT ( 'NONE',  ( -60.31533853284810220, -284.3348481670145134, -197.4306112188495206 ) ) ;
#57719=CARTESIAN_POINT ( 'NONE',  ( 28.28873286595062453, -286.1028890882653286, -305.5985316601507975 ) ) ;
#57720=CARTESIAN_POINT ( 'NONE',  ( -3.259187464325852268, -278.4673666485829244, -338.0415642729728916 ) ) ;
#57721=CARTESIAN_POINT ( 'NONE',  ( -102.0511510180885324, -273.3470576681523880, -236.4170738947551058 ) ) ;
#57723=CARTESIAN_POINT ( 'NONE',  ( 20.06856784116714820, -292.8810005181583733, -316.2647719631617633 ) ) ;
#57724=CARTESIAN_POINT ( 'NONE',  ( -109.1321013365486721, -278.7267303806183349, -257.1271354252457968 ) ) ;
#57725=CARTESIAN_POINT ( 'NONE',  ( -64.84678789747771077, -279.0317420668911268, -202.6310447866929962 ) ) ;
#57726=CARTESIAN_POINT ( 'NONE',  ( -10.46886258239271861, -275.4742251133558852, -198.4760590332703600 ) ) ;
#57727=CARTESIAN_POINT ( 'NONE',  ( -112.9099897138440411, -277.1893420362796974, -282.9087204638536832 ) ) ;
#57728=CARTESIAN_POINT ( 'NONE',  ( 187.5403984051958730, 270.4479071988321266, -138.3868815421773490 ) ) ;
#57729=CARTESIAN_POINT ( 'NONE',  ( -113.0661588182869934, -297.8437671998181600, -280.9662061453626052 ) ) ;
#57730=CARTESIAN_POINT ( 'NONE',  ( 10.59707575819634329, -277.1948066931274184, -210.1954327657594490 ) ) ;
#57732=CARTESIAN_POINT ( 'NONE',  ( 82.67702266595013327, -297.3455801312759377, -194.1454284809947524 ) ) ;
#57734=CARTESIAN_POINT ( 'NONE',  ( -85.94131213312373063, -286.4399162487915760, -215.4087993453869956 ) ) ;
#57735=CARTESIAN_POINT ( 'NONE',  ( -84.89641334288039332, -287.1665508542258749, -211.0945737747394730 ) ) ;
#57736=CARTESIAN_POINT ( 'NONE',  ( -15.82956068846278264, -288.1151215027998092, -340.2790312140961078 ) ) ;
#57737=CARTESIAN_POINT ( 'NONE',  ( -105.3747458795350269, -284.5253879910842443, -234.3161349197571326 ) ) ;
#57738=CARTESIAN_POINT ( 'NONE',  ( 3.159868899270529496, -279.0056476542673067, -208.6064873102757531 ) ) ;
#57739=CARTESIAN_POINT ( 'NONE',  ( -72.98759480476644512, -287.4349761001529941, -205.2295667998179738 ) ) ;
#57740=CARTESIAN_POINT ( 'NONE',  ( 34.90661833087635557, -280.2226230419719855, -284.9465326302661197 ) ) ;
#57741=CARTESIAN_POINT ( 'NONE',  ( -73.06717479543813454, -278.8513544616861282, -334.6012439097072502 ) ) ;
#57742=CARTESIAN_POINT ( 'NONE',  ( 33.95469671935499179, -276.2556496899053400, -286.3808676455569753 ) ) ;
#57743=CARTESIAN_POINT ( 'NONE',  ( -59.92493121506618081, -288.1333826715351165, -343.5595222778960647 ) ) ;
#57745=CARTESIAN_POINT ( 'NONE',  ( -69.11033991755203942, -284.2622764521086083, -340.3391509866131059 ) ) ;
#57746=CARTESIAN_POINT ( 'NONE',  ( -2.914747351707708489, -283.1018153499184677, -339.1820956484730800 ) ) ;
#57749=CARTESIAN_POINT ( 'NONE',  ( 4.888799411908724579, -290.3485496442762042, -333.2649365250067035 ) ) ;
#57751=CARTESIAN_POINT ( 'NONE',  ( -111.8332570173745779, -289.4565636170700031, -252.9167427499722294 ) ) ;
#57752=CARTESIAN_POINT ( 'NONE',  ( -107.4181753083423132, -271.8937865218068737, -248.9108431243769530 ) ) ;
#57753=CARTESIAN_POINT ( 'NONE',  ( 32.09749340807007201, -292.4753092350247243, -237.1993157039026698 ) ) ;
#57754=CARTESIAN_POINT ( 'NONE',  ( -110.9368534842396912, -289.0932929339947464, -265.6723955499365957 ) ) ;
#57755=CARTESIAN_POINT ( 'NONE',  ( 29.29729805209579041, -292.2232980844642611, -302.6851045285180248 ) ) ;
#57756=CARTESIAN_POINT ( 'NONE',  ( 34.95582976941094699, -288.5874122432589388, -257.4178429492077385 ) ) ;
#57757=CARTESIAN_POINT ( 'NONE',  ( 31.98288692825981272, -290.4805209788416391, -303.7098442033569654 ) ) ;
#57758=CARTESIAN_POINT ( 'NONE',  ( -12.85207459233313720, -290.7341651388443893, -341.3046064698045825 ) ) ;
#57759=CARTESIAN_POINT ( 'NONE',  ( -112.4213510695021938, -288.5056641635710548, -273.9769772615578631 ) ) ;
#57760=CARTESIAN_POINT ( 'NONE',  ( -7.664778281854705000, -294.4412563172717796, -201.4686707104418701 ) ) ;
#57761=CARTESIAN_POINT ( 'NONE',  ( -109.2080877495406952, -285.3080857496458975, -284.4547611934959264 ) ) ;
#57762=CARTESIAN_POINT ( 'NONE',  ( -40.57956414041738213, -294.0117071850597767, -195.2513479720633711 ) ) ;
#57763=CARTESIAN_POINT ( 'NONE',  ( -112.7464469908924372, -270.5823899088603071, -270.3360381906339853 ) ) ;
#57766=CARTESIAN_POINT ( 'NONE',  ( -86.97243596677564881, -275.3456628214781290, -213.5890167831123279 ) ) ;
#57767=CARTESIAN_POINT ( 'NONE',  ( 32.38209641834988162, -281.0444801106273189, -292.6889342037769097 ) ) ;
#57768=CARTESIAN_POINT ( 'NONE',  ( -68.64163157441971919, -281.4633582630633555, -338.5176653127900863 ) ) ;
#57769=CARTESIAN_POINT ( 'NONE',  ( -61.55040797592001667, -294.5558722014347950, -343.3420285469898090 ) ) ;
#57770=CARTESIAN_POINT ( 'NONE',  ( -18.99911030312427940, -272.5312068727891983, -198.6035421330635415 ) ) ;
#57771=CARTESIAN_POINT ( 'NONE',  ( -74.75780986872122469, -275.6342255996005406, -334.7144312626272153 ) ) ;
#57772=CARTESIAN_POINT ( 'NONE',  ( -109.5332298730474179, -298.0486455991762114, -256.5235197740528861 ) ) ;
#57773=CARTESIAN_POINT ( 'NONE',  ( 35.05965138847447804, -294.8041841703094974, -257.1222685173057698 ) ) ;
#57776=CARTESIAN_POINT ( 'NONE',  ( -20.80175114107759526, -295.6373455389812079, -341.6806661967788159 ) ) ;
#57778=CARTESIAN_POINT ( 'NONE',  ( 35.89966613158416209, -285.7994174933493241, -288.1386740624200797 ) ) ;
#57779=CARTESIAN_POINT ( 'NONE',  ( -99.89679438943502987, -297.0710668442935685, -232.6348975792506337 ) ) ;
#57780=CARTESIAN_POINT ( 'NONE',  ( -106.6791117930616082, -284.9817943683661383, -236.8749515313063796 ) ) ;
#57781=CARTESIAN_POINT ( 'NONE',  ( 39.61900482242741361, -287.1979604971948561, -268.6895364089406826 ) ) ;
#57782=CARTESIAN_POINT ( 'NONE',  ( -52.92396907888562652, -297.2306657816783968, -344.1410116829302410 ) ) ;
#57783=CARTESIAN_POINT ( 'NONE',  ( 36.01866337056321754, -291.3618678655024041, -255.5866299321801307 ) ) ;
#57784=CARTESIAN_POINT ( 'NONE',  ( -108.3595099276998326, -278.1229718434256029, -241.0246302697951251 ) ) ;
#57786=CARTESIAN_POINT ( 'NONE',  ( -4.402680322401938184, -285.2912578954010314, -204.7703299076844985 ) ) ;
#57787=CARTESIAN_POINT ( 'NONE',  ( -97.92391466445977244, -288.8419787091631861, -317.3854499074386695 ) ) ;
#57790=CARTESIAN_POINT ( 'NONE',  ( -108.9561560288349256, -298.3855953646112198, -252.4820924810838960 ) ) ;
#57791=CARTESIAN_POINT ( 'NONE',  ( -68.44939123727516517, -281.0766820065049956, -200.5548793429686327 ) ) ;
#57792=CARTESIAN_POINT ( 'NONE',  ( -105.0246925091827563, -295.0069644303174528, -237.2337978060400587 ) ) ;
#57793=CARTESIAN_POINT ( 'NONE',  ( 28.99366614562987365, -280.8057480637577328, -239.7160552336791568 ) ) ;
#57794=CARTESIAN_POINT ( 'NONE',  ( -13.78002624022826161, -294.9212698721096899, -343.6676492611216531 ) ) ;
#57796=CARTESIAN_POINT ( 'NONE',  ( -110.7649813417112341, -280.7495242602191752, -255.0012891508309849 ) ) ;
#57797=CARTESIAN_POINT ( 'NONE',  ( -108.8241415588536398, -295.4014697618312653, -286.2881081576207976 ) ) ;
#57801=CARTESIAN_POINT ( 'NONE',  ( -45.80138954890485792, -285.1396813555134031, -344.5771354168640528 ) ) ;
#57803=CARTESIAN_POINT ( 'NONE',  ( -106.6379572354042296, -282.4809262143061233, -236.9535640164627353 ) ) ;
#57804=CARTESIAN_POINT ( 'NONE',  ( 5.772212440723139437, -275.6810090601581464, -333.9641789397207958 ) ) ;
#57805=CARTESIAN_POINT ( 'NONE',  ( -41.59071488508229919, -291.8306081738162447, -197.4350347343781493 ) ) ;
#57806=CARTESIAN_POINT ( 'NONE',  ( 36.25934914640646411, -283.1204603871029235, -274.0480267787647790 ) ) ;
#57807=CARTESIAN_POINT ( 'NONE',  ( -1.350090298528437760, -276.1380331527329872, -205.9180500180696356 ) ) ;
#57808=CARTESIAN_POINT ( 'NONE',  ( -13.65111067311097592, -284.3497717476746516, -342.7848460376803814 ) ) ;
#57809=CARTESIAN_POINT ( 'NONE',  ( 33.12006312800805574, -280.0767053996023037, -249.8118984309327004 ) ) ;
#57810=CARTESIAN_POINT ( 'NONE',  ( -109.7445322865349482, -280.3007506770264854, -289.9271739634959317 ) ) ;
#57811=CARTESIAN_POINT ( 'NONE',  ( -114.3417001280813849, -272.7188053819918423, -270.3632355433240946 ) ) ;
#57812=CARTESIAN_POINT ( 'NONE',  ( 31.25125891221065899, -274.9348930203797181, -235.3753212275701401 ) ) ;
#57813=CARTESIAN_POINT ( 'NONE',  ( 24.13579854213000075, -296.0460874053790121, -312.4254733604076932 ) ) ;
#57815=DIRECTION ( 'NONE',  ( -1.000000000000000000, -0.000000000000000000, -0.000000000000000000 ) ) ;
#57816=CARTESIAN_POINT ( 'NONE',  ( 1.121622863161765293, -292.6839494628433158, -335.6365211972881752 ) ) ;
#57817=CARTESIAN_POINT ( 'NONE',  ( -64.58591646424200405, -273.1942962258875696, -202.5557316824814507 ) ) ;
#57818=CARTESIAN_POINT ( 'NONE',  ( -44.84828177921385617, -293.4790213086195649, -194.3721261434434666 ) ) ;
#57819=CARTESIAN_POINT ( 'NONE',  ( -110.4683760289727132, -281.2662352645559167, -253.7030783399848985 ) ) ;
#57820=CARTESIAN_POINT ( 'NONE',  ( -25.10009313219005733, -293.4100133111776358, -194.7426561111478520 ) ) ;
#57821=CARTESIAN_POINT ( 'NONE',  ( -15.28763104685571150, -290.7662682559471250, -341.9250413499781871 ) ) ;
#57822=CARTESIAN_POINT ( 'NONE',  ( -111.0972525387210084, -276.3881652039447090, -283.0919244991044934 ) ) ;
#57823=CARTESIAN_POINT ( 'NONE',  ( -71.08409885277004037, -279.4212488446241309, -336.7144504479687726 ) ) ;
#57824=CARTESIAN_POINT ( 'NONE',  ( 35.36140050471799157, -291.4244242868235233, -254.3154287362765444 ) ) ;
#57825=CARTESIAN_POINT ( 'NONE',  ( 35.78647983263250154, -283.1598202765108567, -250.4984772312153325 ) ) ;
#57826=CARTESIAN_POINT ( 'NONE',  ( -94.53477287839518794, -282.8269493298037105, -316.2415165367745544 ) ) ;
#57828=CARTESIAN_POINT ( 'NONE',  ( -34.85006969594519433, -282.6867461291899986, -343.3521801830165145 ) ) ;
#57829=CARTESIAN_POINT ( 'NONE',  ( 18.92399340976638200, -281.9190673254566946, -218.2490825153763296 ) ) ;
#57830=CARTESIAN_POINT ( 'NONE',  ( -105.4382413256048636, -282.8912557907726750, -305.5606529913536633 ) ) ;
#57831=CARTESIAN_POINT ( 'NONE',  ( -79.79068279718737244, -280.4349750822498777, -206.3371713435682295 ) ) ;
#57832=CARTESIAN_POINT ( 'NONE',  ( 37.50610666046531350, -277.2596719233403064, -285.2108174230646682 ) ) ;
#57833=CARTESIAN_POINT ( 'NONE',  ( -102.0455923789670294, -275.6237833571633473, -301.4846348637937581 ) ) ;
#57834=ORIENTED_EDGE ( 'NONE', *, *, #51060, .T. ) ;
#57835=ORIENTED_EDGE ( 'NONE', *, *, #41133, .T. ) ;
#57836=CARTESIAN_POINT ( 'NONE',  ( -112.0201622706384086, -274.6238543458640606, -264.8020081627651621 ) ) ;
#57837=CARTESIAN_POINT ( 'NONE',  ( -72.44959466576179352, -275.5392528130773258, -336.2487682997601723 ) ) ;
#57838=CARTESIAN_POINT ( 'NONE',  ( -106.3496901585683929, -292.7260543352621767, -238.4257486068886749 ) ) ;
#57839=CARTESIAN_POINT ( 'NONE',  ( -4.297994806941224155, -293.9532431717657914, -335.5825442155469887 ) ) ;
#57840=CARTESIAN_POINT ( 'NONE',  ( -113.6042835426848256, -290.1920487732495531, -259.7955929139251339 ) ) ;
#57842=CARTESIAN_POINT ( 'NONE',  ( 38.91277767054699410, -292.1981209500998489, -276.0137753120155821 ) ) ;
#57843=CARTESIAN_POINT ( 'NONE',  ( -93.85471623216888304, -283.6187702111141675, -222.8982964493575594 ) ) ;
#57844=CARTESIAN_POINT ( 'NONE',  ( -64.54595376625732683, -293.5536543824113664, -201.2764188900407873 ) ) ;
#57845=CARTESIAN_POINT ( 'NONE',  ( 0.5415417606193264621, -285.0464291341202738, -207.0911145497513814 ) ) ;
#57846=CARTESIAN_POINT ( 'NONE',  ( 16.19652850644765607, -283.5879298208346881, -320.7823645135568427 ) ) ;
#57847=CARTESIAN_POINT ( 'NONE',  ( -113.8768577201574885, -291.4108045686492119, -276.9453784949673150 ) ) ;
#57848=CARTESIAN_POINT ( 'NONE',  ( -32.96558757828728403, -280.6011196102725762, -197.4307533824961070 ) ) ;
#57849=CARTESIAN_POINT ( 'NONE',  ( -4.685806924308310251, -293.4264445389100615, -339.6690997346877907 ) ) ;
#57850=CARTESIAN_POINT ( 'NONE',  ( 24.01944054576840060, -288.9721099633155177, -316.6101097146308803 ) ) ;
#57851=CARTESIAN_POINT ( 'NONE',  ( 10.19485166872850002, -288.9090950637611286, -330.9252065908653435 ) ) ;
#57852=CARTESIAN_POINT ( 'NONE',  ( -27.83865374061423381, -286.3428745546037248, -197.9823081425884936 ) ) ;
#57853=VERTEX_POINT ( 'NONE', #68990 ) ;
#57855=CARTESIAN_POINT ( 'NONE',  ( -0.04654210041249363938, -296.4218478209982095, -336.3258605110382291 ) ) ;
#57856=CARTESIAN_POINT ( 'NONE',  ( -111.4948433797446654, -294.9992302148526164, -289.2451344136368334 ) ) ;
#57857=CARTESIAN_POINT ( 'NONE',  ( -92.37736379734205627, -278.2985208206132484, -222.0255447989806328 ) ) ;
#57858=CARTESIAN_POINT ( 'NONE',  ( -49.70316693167568900, -273.4063302281891765, -194.3684263932130420 ) ) ;
#57859=CARTESIAN_POINT ( 'NONE',  ( -28.83498333370479116, -293.4223662025949579, -343.6133221923825545 ) ) ;
#57860=CARTESIAN_POINT ( 'NONE',  ( 22.28441923346398923, -276.7063135000776128, -226.5125158938447498 ) ) ;
#57861=CARTESIAN_POINT ( 'NONE',  ( -74.87783365778203404, -271.6866688751387073, -206.2554713857131787 ) ) ;
#57862=CARTESIAN_POINT ( 'NONE',  ( 33.00526069309908195, -294.4795374805362940, -249.2472545493952225 ) ) ;
#57863=CARTESIAN_POINT ( 'NONE',  ( -7.851396289375895066, -295.7360905516576395, -337.4906842188781297 ) ) ;
#57865=VECTOR ( 'NONE', #42987, 1000.000000000000000 ) ;
#57866=CARTESIAN_POINT ( 'NONE',  ( -110.5268021382999279, -294.3316239338815308, -287.5624013188418644 ) ) ;
#57867=CARTESIAN_POINT ( 'NONE',  ( 76.19145359092561876, -300.0900639254019779, -193.4507982650258384 ) ) ;
#57868=CARTESIAN_POINT ( 'NONE',  ( -102.4667466277641665, -275.0496087501944658, -233.0581151396938822 ) ) ;
#57869=CARTESIAN_POINT ( 'NONE',  ( -109.4083297353386968, -291.3220579673526913, -283.3922094802898641 ) ) ;
#57871=CARTESIAN_POINT ( 'NONE',  ( 1.584694542675792572, -294.8497020746069666, -332.2014491539438268 ) ) ;
#57873=CARTESIAN_POINT ( 'NONE',  ( -103.3648796476223879, -281.0127494249105666, -234.0383074317571186 ) ) ;
#57874=CARTESIAN_POINT ( 'NONE',  ( -101.4686624080805046, -277.7896127248654921, -228.5396223160616671 ) ) ;
#57875=CARTESIAN_POINT ( 'NONE',  ( -4.215270454074896200, -281.9754406002269320, -339.7726506801226378 ) ) ;
#57876=CARTESIAN_POINT ( 'NONE',  ( 37.84747674733428369, -274.6980745747902688, -254.1774086232588843 ) ) ;
#57877=CARTESIAN_POINT ( 'NONE',  ( -36.73820986990828175, -278.4594963937113903, -194.1505946666885336 ) ) ;
#57878=CARTESIAN_POINT ( 'NONE',  ( -9.515542739389985627, -278.4147702630452272, -200.5346660301104009 ) ) ;
#57880=CARTESIAN_POINT ( 'NONE',  ( -44.60124279313166795, -296.6433344707083393, -197.1766654755183765 ) ) ;
#57881=CARTESIAN_POINT ( 'NONE',  ( -3.143706023520141279, -278.6006310360558018, -337.1247252722678240 ) ) ;
#57883=CARTESIAN_POINT ( 'NONE',  ( -80.54061425516390216, -289.6198778182628644, -334.1660497808048262 ) ) ;
#57884=CARTESIAN_POINT ( 'NONE',  ( 1.449535284803833424, -276.5694342071365099, -205.9773585294363443 ) ) ;
#57885=CARTESIAN_POINT ( 'NONE',  ( -68.79545319683467142, -295.6375985316801689, -202.4450512996676821 ) ) ;
#57886=CARTESIAN_POINT ( 'NONE',  ( -114.1647661948828443, -283.7900534034688462, -267.1110178693853072 ) ) ;
#57888=CARTESIAN_POINT ( 'NONE',  ( -107.4669790830532179, -282.2047231629902626, -297.1033203871699584 ) ) ;
#57890=CARTESIAN_POINT ( 'NONE',  ( 9.111952221624832760, -291.5010449112647279, -213.4692338362773967 ) ) ;
#57891=CARTESIAN_POINT ( 'NONE',  ( -92.42205425272727837, -283.3933965791152900, -220.5159444926252661 ) ) ;
#57894=CARTESIAN_POINT ( 'NONE',  ( -1.460802696476545481, -290.5276815216863611, -204.4863626861958323 ) ) ;
#57895=CARTESIAN_POINT ( 'NONE',  ( -70.18936673350430056, -281.9569427535006412, -339.2502542054396031 ) ) ;
#57896=CARTESIAN_POINT ( 'NONE',  ( -37.79443643331234171, -278.6580090122620277, -344.1723217956323992 ) ) ;
#57897=CARTESIAN_POINT ( 'NONE',  ( -109.8438923513058683, -285.4440442925561001, -295.0884478222125722 ) ) ;
#57898=CARTESIAN_POINT ( 'NONE',  ( 20.34065409041034656, -286.9219765256700043, -225.6202416856829984 ) ) ;
#57899=CARTESIAN_POINT ( 'NONE',  ( -67.02381664825605867, -278.8743147684258474, -337.6986771700387067 ) ) ;
#57900=CARTESIAN_POINT ( 'NONE',  ( -99.30642705152872907, -278.8178961819338042, -309.3526999864703271 ) ) ;
#57903=CARTESIAN_POINT ( 'NONE',  ( -112.1588004300198094, -286.6284405435655458, -264.4323774020255655 ) ) ;
#57905=CARTESIAN_POINT ( 'NONE',  ( -109.8501484178673024, -296.7125833971868474, -244.4473198992276366 ) ) ;
#57906=CARTESIAN_POINT ( 'NONE',  ( -42.75866125769783821, -291.1005951400370577, -344.8608526396287743 ) ) ;
#57908=CARTESIAN_POINT ( 'NONE',  ( -19.05039376806008633, -279.3376638359844719, -350.3538533559490702 ) ) ;
#57910=CARTESIAN_POINT ( 'NONE',  ( 38.80667523918234707, -291.9874672286117629, -273.1656397652747614 ) ) ;
#57911=CARTESIAN_POINT ( 'NONE',  ( 9.456007311339179822, -288.2294416836294886, -213.4341267663791371 ) ) ;
#57912=CARTESIAN_POINT ( 'NONE',  ( 15.97399349310584959, -282.5804604705991778, -218.9516753940150693 ) ) ;
#57913=CARTESIAN_POINT ( 'NONE',  ( 22.51886840566906400, -288.3367686659740343, -222.8500748988525118 ) ) ;
#57914=CARTESIAN_POINT ( 'NONE',  ( 20.21304111122029923, -289.5538065796483806, -320.7867128219516530 ) ) ;
#57915=CARTESIAN_POINT ( 'NONE',  ( -108.0510130008192817, -286.2266261893999513, -295.5194913067584253 ) ) ;
#57916=CARTESIAN_POINT ( 'NONE',  ( -112.1746771988216977, -278.4912865205049570, -288.5553989295952420 ) ) ;
#57918=CARTESIAN_POINT ( 'NONE',  ( -66.39380901124575018, -293.5094113721327744, -340.1266812087301332 ) ) ;
#57919=CARTESIAN_POINT ( 'NONE',  ( 39.61973873679414027, -281.4159453059051543, -272.7977000832070189 ) ) ;
#57921=CARTESIAN_POINT ( 'NONE',  ( -111.1158943255973952, -274.5197282854189780, -262.1007457237456038 ) ) ;
#57923=CARTESIAN_POINT ( 'NONE',  ( -20.19161114001083490, -285.3376638359844719, -345.3538533559490702 ) ) ;
#57924=CARTESIAN_POINT ( 'NONE',  ( -68.40898256894826091, -271.8894786957691849, -201.0014173510717796 ) ) ;
#57927=CARTESIAN_POINT ( 'NONE',  ( -98.04124089976497203, -278.6252053204775052, -229.6073770932732998 ) ) ;
#57929=CARTESIAN_POINT ( 'NONE',  ( 36.11707773595592386, -277.0316649527828190, -292.1287710924053727 ) ) ;
#57930=CARTESIAN_POINT ( 'NONE',  ( -110.6821377199610623, -273.9389781816997242, -264.8933313537352774 ) ) ;
#57931=CARTESIAN_POINT ( 'NONE',  ( -66.49801737263513246, -282.4835095047158688, -341.3874393040812265 ) ) ;
#57932=CARTESIAN_POINT ( 'NONE',  ( -110.1721191573525260, -292.1408148815614254, -283.5408023120857592 ) ) ;
#57933=CARTESIAN_POINT ( 'NONE',  ( -77.85093423925658840, -299.0385433309144787, -205.6949776643984364 ) ) ;
#57935=CARTESIAN_POINT ( 'NONE',  ( -31.95972564808470651, -299.3231944964703075, -193.7571136113821808 ) ) ;
#57936=CARTESIAN_POINT ( 'NONE',  ( -2.262357959318330725, -296.5868824734182567, -336.4630709188574542 ) ) ;
#57937=CARTESIAN_POINT ( 'NONE',  ( -111.3144852122869821, -282.4020810451276020, -282.0104606228945840 ) ) ;
#57939=CARTESIAN_POINT ( 'NONE',  ( -114.3475782948352872, -290.2440174991040749, -268.3510277801652251 ) ) ;
#57940=CARTESIAN_POINT ( 'NONE',  ( -2.115670954142796489, -272.5410678256044434, -204.5509844656145333 ) ) ;
#57941=CARTESIAN_POINT ( 'NONE',  ( -60.28862596415066122, -287.3597616271641755, -197.6433379493414861 ) ) ;
#57942=CARTESIAN_POINT ( 'NONE',  ( -57.72776959917503348, -290.7030995603292922, -199.8904496458704614 ) ) ;
#57943=CARTESIAN_POINT ( 'NONE',  ( 86.00283748409529494, 82.43107403786450504, -302.1230288021248498 ) ) ;
#57945=CARTESIAN_POINT ( 'NONE',  ( -112.2936024482960562, -288.9387711388957882, -285.2874840546044766 ) ) ;
#57946=CARTESIAN_POINT ( 'NONE',  ( 23.52477684991707108, -287.7787543665789940, -310.7244985655486289 ) ) ;
#57948=CARTESIAN_POINT ( 'NONE',  ( -63.11056363648066991, -286.8039004798685596, -198.1291431867735753 ) ) ;
#57950=CARTESIAN_POINT ( 'NONE',  ( -24.32166502937336006, -277.2147515623557297, -342.2635838837631468 ) ) ;
#57951=CARTESIAN_POINT ( 'NONE',  ( 34.15832040752763987, -292.8252844319943051, -298.0962864966012944 ) ) ;
#57952=CARTESIAN_POINT ( 'NONE',  ( -34.47445531282367170, -283.6684072047224277, -347.2057124185507746 ) ) ;
#57953=CARTESIAN_POINT ( 'NONE',  ( -67.58856242056587860, -284.9619679137530284, -340.4170604531349227 ) ) ;
#57954=CARTESIAN_POINT ( 'NONE',  ( -83.86704695503310347, -284.0044684746486610, -331.7561795584875313 ) ) ;
#57955=CARTESIAN_POINT ( 'NONE',  ( 25.15218519376723449, -281.3645076886259631, -232.4927573085191455 ) ) ;
#57956=CARTESIAN_POINT ( 'NONE',  ( -104.2036854529545877, -256.2936084490758049, -326.7685368105336465 ) ) ;
#57957=CARTESIAN_POINT ( 'NONE',  ( 152.5227351927868824, 207.2448686218533851, -216.6814332530730667 ) ) ;
#57958=CARTESIAN_POINT ( 'NONE',  ( -99.20933047681515404, -245.9584877323212879, -331.5210257661068454 ) ) ;
#57960=CARTESIAN_POINT ( 'NONE',  ( -21.88997815373728884, -273.4524329690652849, -198.8499579133226973 ) ) ;
#57961=CARTESIAN_POINT ( 'NONE',  ( -103.0662753845434594, -295.5371147025082905, -310.3587067909311372 ) ) ;
#57962=CARTESIAN_POINT ( 'NONE',  ( 65.87130157267131381, 45.95421370783718373, -315.7040055182292804 ) ) ;
#57963=CARTESIAN_POINT ( 'NONE',  ( -83.27058146805659078, -272.1228470166442435, -209.1079281782014050 ) ) ;
#57964=CARTESIAN_POINT ( 'NONE',  ( -105.9120666866129881, -298.7876250773315405, -241.9187146393726664 ) ) ;
#57965=CARTESIAN_POINT ( 'NONE',  ( 35.61577882131522443, -288.9833888269830595, -279.2183039413944243 ) ) ;
#57967=CARTESIAN_POINT ( 'NONE',  ( -58.77409896342661000, -296.2638914781307449, -344.1286095331149113 ) ) ;
#57968=CARTESIAN_POINT ( 'NONE',  ( -85.77162586964622903, -285.8526865714146652, -215.5894649151744318 ) ) ;
#57969=CARTESIAN_POINT ( 'NONE',  ( -31.27076875955219037, -273.0474397133080515, -193.8976688145276057 ) ) ;
#57971=CARTESIAN_POINT ( 'NONE',  ( 11.10444422333766212, -295.2040053080797293, -330.0713715905176286 ) ) ;
#57972=CARTESIAN_POINT ( 'NONE',  ( 15.44102743755717455, -294.8219663328866318, -326.3388865504052205 ) ) ;
#57973=CARTESIAN_POINT ( 'NONE',  ( -109.7892537389686822, -290.6005840244441742, -279.3250445941597491 ) ) ;
#57974=ORIENTED_EDGE ( 'NONE', *, *, #59748, .F. ) ;
#57975=CARTESIAN_POINT ( 'NONE',  ( -36.97180572203875926, -275.9769297164795034, -194.7892118385888409 ) ) ;
#57976=CARTESIAN_POINT ( 'NONE',  ( 25.82587467193739172, -273.7719727846267119, -227.0035082255900818 ) ) ;
#57979=CARTESIAN_POINT ( 'NONE',  ( -112.7345878779304655, -277.8669404598197161, -285.7702861374085046 ) ) ;
#57981=CARTESIAN_POINT ( 'NONE',  ( -1.314477122054709790, -272.9382931443856819, -205.9379537215812945 ) ) ;
#57982=CARTESIAN_POINT ( 'NONE',  ( -90.42990050973847360, -274.3579567062921001, -219.7871448756984023 ) ) ;
#57983=CARTESIAN_POINT ( 'NONE',  ( 33.81800032064830219, -276.7217166434894011, -287.7259852466841039 ) ) ;
#57984=CARTESIAN_POINT ( 'NONE',  ( -36.21977334332840570, -299.6660977551940164, -194.1608129806244563 ) ) ;
#57985=CARTESIAN_POINT ( 'NONE',  ( 35.98536907922287753, -273.7948330341387191, -287.7817467990586238 ) ) ;
#57986=CARTESIAN_POINT ( 'NONE',  ( -108.9829614058983935, -297.0112024697855873, -284.9637921210493232 ) ) ;
#57987=CARTESIAN_POINT ( 'NONE',  ( 35.29848094363444488, -291.9716832778467506, -258.5017518920986390 ) ) ;
#57989=CARTESIAN_POINT ( 'NONE',  ( -97.87660440787995242, -278.4091601258947435, -317.8485085972333195 ) ) ;
#57990=CARTESIAN_POINT ( 'NONE',  ( 35.37801293613929943, -275.6272503179661726, -263.4186342899220676 ) ) ;
#57991=CARTESIAN_POINT ( 'NONE',  ( -85.19136032609551989, -284.0917305533400850, -210.6643149663782140 ) ) ;
#57992=CARTESIAN_POINT ( 'NONE',  ( -111.7895985030628623, -298.6863644335945196, -259.8976917860873641 ) ) ;
#57995=CARTESIAN_POINT ( 'NONE',  ( 4.826764251499326974, -285.8349637300727863, -210.5126447686693041 ) ) ;
#57996=CARTESIAN_POINT ( 'NONE',  ( -97.72523120260932217, -276.2023397483587814, -313.1827078333365648 ) ) ;
#57997=CARTESIAN_POINT ( 'NONE',  ( -109.0646139898000655, -276.9106445390127647, -286.8851283024349073 ) ) ;
#57998=CARTESIAN_POINT ( 'NONE',  ( -52.99558996750827333, -285.2528415699865718, -343.7617614044169727 ) ) ;
#57999=CARTESIAN_POINT ( 'NONE',  ( -78.84395163397067563, -278.8300969374211604, -330.9597099508901010 ) ) ;
#58002=CARTESIAN_POINT ( 'NONE',  ( 31.83544251731552066, -273.5375228602582638, -238.2828760193348785 ) ) ;
#58004=CARTESIAN_POINT ( 'NONE',  ( -11.46188540723281157, -275.0496619549842308, -201.9394054434694397 ) ) ;
#58005=CARTESIAN_POINT ( 'NONE',  ( -4.482612943415483109, -282.4842437346626980, -202.7428891052908568 ) ) ;
#58007=CARTESIAN_POINT ( 'NONE',  ( -8.754838620703363716, -290.6012186759199949, -340.3187079258790959 ) ) ;
#58008=CARTESIAN_POINT ( 'NONE',  ( -5.114983384847434422, -290.4761587534719638, -202.6239211019535276 ) ) ;
#58010=CARTESIAN_POINT ( 'NONE',  ( -47.31157739077964663, -296.7177062594981294, -197.5928365763701891 ) ) ;
#58011=CARTESIAN_POINT ( 'NONE',  ( -108.9369993599405575, -288.9466569878051132, -250.7402461863096903 ) ) ;
#58012=CARTESIAN_POINT ( 'NONE',  ( 206.7397234113112461, 289.2571863808457238, -82.84736978277094011 ) ) ;
#58014=CARTESIAN_POINT ( 'NONE',  ( -97.62389091526596019, -288.4015994249926962, -317.1453592308348561 ) ) ;
#58015=CARTESIAN_POINT ( 'NONE',  ( 3.853494484154238897, -284.0878342660837461, -331.6552591172966800 ) ) ;
#58016=CARTESIAN_POINT ( 'NONE',  ( -69.34535327703582652, -283.8767370577998008, -201.4285841878118504 ) ) ;
#58018=CARTESIAN_POINT ( 'NONE',  ( -38.87933752907440521, -284.4970543968106540, -343.9468747881980448 ) ) ;
#58019=CARTESIAN_POINT ( 'NONE',  ( -92.67456725497034142, -284.6743141904848926, -318.2432709669318456 ) ) ;
#58020=CARTESIAN_POINT ( 'NONE',  ( -95.32966075447173182, -293.1933996588815035, -222.2183753510427664 ) ) ;
#58021=CARTESIAN_POINT ( 'NONE',  ( -21.36332248027393277, -274.5849746800601565, -195.0588222726696017 ) ) ;
#58022=AXIS2_PLACEMENT_3D ( 'NONE', #66171, #22587, #50074 ) ;
#58023=CARTESIAN_POINT ( 'NONE',  ( -110.8672560792099517, -288.4093398246986339, -287.8322593850211888 ) ) ;
#58024=CARTESIAN_POINT ( 'NONE',  ( -89.21211456894610592, -277.7584503748461771, -327.2685876656598793 ) ) ;
#58025=CARTESIAN_POINT ( 'NONE',  ( -15.07875183164729904, -296.7424399670423441, -341.6630050940867704 ) ) ;
#58027=CARTESIAN_POINT ( 'NONE',  ( -95.99890600148557951, -293.6948066931273615, -223.6242672951989618 ) ) ;
#58028=CARTESIAN_POINT ( 'NONE',  ( -7.065519761082431849, -281.3312207024949885, -337.3420515909402297 ) ) ;
#58029=CARTESIAN_POINT ( 'NONE',  ( -112.2543317963196756, -276.4651448884366118, -277.1397823103512792 ) ) ;
#58030=CARTESIAN_POINT ( 'NONE',  ( -87.56534430447884176, -271.8462119899706977, -212.8427033253181833 ) ) ;
#58031=CARTESIAN_POINT ( 'NONE',  ( 32.19258364702903208, -275.1996099819655228, -292.9193991244355857 ) ) ;
#58032=CARTESIAN_POINT ( 'NONE',  ( -30.76418577546842670, -293.6569318120509138, -196.9619077869228931 ) ) ;
#58034=CARTESIAN_POINT ( 'NONE',  ( 6.808581593899909024, -293.6111131926185749, -211.9302950269529902 ) ) ;
#58036=CARTESIAN_POINT ( 'NONE',  ( -27.93973295721343675, -293.5944217172304889, -194.4777209330175651 ) ) ;
#58037=CARTESIAN_POINT ( 'NONE',  ( 38.74846915369588629, -294.9738405522844573, -278.8235739748855622 ) ) ;
#58038=CARTESIAN_POINT ( 'NONE',  ( -109.8047542567639567, -296.2635457049055390, -279.6037386176658970 ) ) ;
#58039=CARTESIAN_POINT ( 'NONE',  ( -75.71797130309303725, -291.5644342604998656, -334.8142557203633487 ) ) ;
#58040=CARTESIAN_POINT ( 'NONE',  ( -69.18451763150262934, -283.6262268035989678, -340.4828423024381436 ) ) ;
#58041=CARTESIAN_POINT ( 'NONE',  ( 19.13128258684973559, -272.9949076995151245, -219.7754980095072312 ) ) ;
#58042=CARTESIAN_POINT ( 'NONE',  ( 1.523511929468046810, -286.3899094786020783, -203.8740162535708578 ) ) ;
#58043=CARTESIAN_POINT ( 'NONE',  ( -71.17631175773820473, -279.4809773108131026, -336.8973176179463280 ) ) ;
#58044=EDGE_CURVE ( 'NONE', #20110, #32677, #69819, .T. ) ;
#58045=CARTESIAN_POINT ( 'NONE',  ( -37.26513326156666039, -284.8480174657229327, -196.9515777883170813 ) ) ;
#58046=CARTESIAN_POINT ( 'NONE',  ( -20.95875266260309644, -286.8418832604791078, -343.6031557897267703 ) ) ;
#58047=CARTESIAN_POINT ( 'NONE',  ( -64.28062463050963515, -277.8440752353067182, -199.4919593508309674 ) ) ;
#58048=CARTESIAN_POINT ( 'NONE',  ( 201.7194887906492795, 294.2213704821156739, -83.28174295417332473 ) ) ;
#58049=CARTESIAN_POINT ( 'NONE',  ( -100.4574440433205496, -283.5551444016153368, -307.1631737887294662 ) ) ;
#58050=CARTESIAN_POINT ( 'NONE',  ( 36.94242822685470173, -282.5219717217978541, -251.6561187980134662 ) ) ;
#58051=CARTESIAN_POINT ( 'NONE',  ( 5.416295624588007840, -287.5473329941611382, -334.1151297126202167 ) ) ;
#58052=CARTESIAN_POINT ( 'NONE',  ( -50.81836651915342884, -281.4828580095158372, -195.3623188151042882 ) ) ;
#58053=CARTESIAN_POINT ( 'NONE',  ( -71.33657836451762080, -278.8068300518057185, -338.9004973820360647 ) ) ;
#58054=CARTESIAN_POINT ( 'NONE',  ( -64.81414821861213227, -279.5163969691662942, -202.7278081387677275 ) ) ;
#58055=CARTESIAN_POINT ( 'NONE',  ( -93.26683097515734744, -275.2227753164444266, -220.9219984096359042 ) ) ;
#58056=CARTESIAN_POINT ( 'NONE',  ( 36.28697950038537812, -293.2691941108852234, -247.8263107686384501 ) ) ;
#58057=CARTESIAN_POINT ( 'NONE',  ( 27.10365975825455109, -286.0790720819892385, -308.1281155714692090 ) ) ;
#58058=CARTESIAN_POINT ( 'NONE',  ( 1.276894379539621260, -294.1586378531939090, -204.6118266236744034 ) ) ;
#58059=CARTESIAN_POINT ( 'NONE',  ( -110.5200336616545087, -295.5299702738424230, -265.9841813721533867 ) ) ;
#58060=CARTESIAN_POINT ( 'NONE',  ( 35.22744216943532081, -293.3317057668817824, -278.9172289681784491 ) ) ;
#58061=CARTESIAN_POINT ( 'NONE',  ( -104.3466099793609629, -292.1174056806706858, -233.0538189002723186 ) ) ;
#58062=CARTESIAN_POINT ( 'NONE',  ( 28.24618613459835004, -282.6417707717410508, -302.7579329370664141 ) ) ;
#58063=CARTESIAN_POINT ( 'NONE',  ( -73.82244513651923512, -272.6389941353839959, -202.7596332637443766 ) ) ;
#58064=CARTESIAN_POINT ( 'NONE',  ( -46.00603543053564692, -289.8105630052190804, -346.8225642779727877 ) ) ;
#58065=CARTESIAN_POINT ( 'NONE',  ( -68.69724718499702476, -281.5994587043184083, -339.3472914433079950 ) ) ;
#58066=CARTESIAN_POINT ( 'NONE',  ( -112.2411303655110117, -290.6624099612610621, -288.1888209112111667 ) ) ;
#58067=CARTESIAN_POINT ( 'NONE',  ( -41.32832582202011906, -286.3338950261834839, -197.4363790608946658 ) ) ;
#58070=CARTESIAN_POINT ( 'NONE',  ( 4.150380923130051691, -57.95720081330512130, -352.8324262869497829 ) ) ;
#58071=CARTESIAN_POINT ( 'NONE',  ( 200.7764005794019226, 290.0384947088795116, -82.33303656482503641 ) ) ;
#58072=CARTESIAN_POINT ( 'NONE',  ( -107.2739951928463853, -277.4631946985408035, -292.0267890297669737 ) ) ;
#58073=CARTESIAN_POINT ( 'NONE',  ( -9.115677510991886834, -279.3504792048175887, -202.7037627185481199 ) ) ;
#58074=CARTESIAN_POINT ( 'NONE',  ( 37.26578296297303439, -274.9815630207957042, -251.4014830062171200 ) ) ;
#58075=CARTESIAN_POINT ( 'NONE',  ( -61.34299255263732675, -183.7475365659067279, -360.0278117845444399 ) ) ;
#58076=CARTESIAN_POINT ( 'NONE',  ( -50.81774693757084549, -278.4579443672043908, -195.1480708842843512 ) ) ;
#58078=CARTESIAN_POINT ( 'NONE',  ( -23.79109945897418044, -280.8982609153710541, -343.7656683956664097 ) ) ;
#58079=CARTESIAN_POINT ( 'NONE',  ( -34.86492208978587115, -296.7815727770631611, -346.3074120756865000 ) ) ;
#58080=CARTESIAN_POINT ( 'NONE',  ( -69.04997580472544882, -292.1159276326052918, -204.5250139924184509 ) ) ;
#58081=CARTESIAN_POINT ( 'NONE',  ( -82.86476396339747907, -288.3748244922185791, -328.0576875132261421 ) ) ;
#58082=CARTESIAN_POINT ( 'NONE',  ( 37.53375497045848164, -275.9834968945108358, -252.7830485950662762 ) ) ;
#58083=CARTESIAN_POINT ( 'NONE',  ( -103.9357459632928169, -296.3145401263366807, -300.3884054730339699 ) ) ;
#58089=CARTESIAN_POINT ( 'NONE',  ( -104.8992630881107289, -280.9172392771650948, -236.4023818595052830 ) ) ;
#58091=CARTESIAN_POINT ( 'NONE',  ( -7.887817190267499612, -281.5270496202666095, -203.2154677488197194 ) ) ;
#58092=CARTESIAN_POINT ( 'NONE',  ( -81.66617511274853314, -281.2179399937946300, -208.6414701474983815 ) ) ;
#58093=CARTESIAN_POINT ( 'NONE',  ( 34.93384275606230460, -280.7662886490513756, -282.1786621100433763 ) ) ;
#58094=CARTESIAN_POINT ( 'NONE',  ( -0.1800722102555995519, -273.0359436540743445, -206.7089669986499985 ) ) ;
#58099=CARTESIAN_POINT ( 'NONE',  ( 37.43709352827445969, -276.5771073813437511, -288.0895771496482780 ) ) ;
#58103=CARTESIAN_POINT ( 'NONE',  ( 37.32359682799047818, -277.4546810761565894, -262.7571168176075389 ) ) ;
#58104=CARTESIAN_POINT ( 'NONE',  ( -42.78246696935688931, -275.6942774959569533, -346.5779425637010149 ) ) ;
#58107=CARTESIAN_POINT ( 'NONE',  ( -108.6596969937836121, -286.2187358259548091, -294.6952529583228397 ) ) ;
#58108=CARTESIAN_POINT ( 'NONE',  ( 27.63462644800139500, -292.2930568541190723, -236.7355516509282438 ) ) ;
#58109=CARTESIAN_POINT ( 'NONE',  ( -7.375185896956212517, -285.7833848721528511, -199.4856045071344965 ) ) ;
#58110=CARTESIAN_POINT ( 'NONE',  ( -59.26944187115613261, -281.5796180740320551, -341.1055124302971535 ) ) ;
#58111=CARTESIAN_POINT ( 'NONE',  ( -29.39895045103452986, -281.5244370202834148, -343.5713594295870053 ) ) ;
#58112=CARTESIAN_POINT ( 'NONE',  ( -11.49959828440748844, -284.4712449703861807, -200.5506605292513314 ) ) ;
#58113=CARTESIAN_POINT ( 'NONE',  ( -40.23472935808855055, -284.2944036596261981, -343.7011540307281621 ) ) ;
#58114=CARTESIAN_POINT ( 'NONE',  ( 28.21215188203397162, -273.0658602033119564, -233.8167363385458941 ) ) ;
#58115=CARTESIAN_POINT ( 'NONE',  ( -107.1846265291710267, -283.3460619258278825, -239.7595096511194015 ) ) ;
#58116=CARTESIAN_POINT ( 'NONE',  ( -44.57666132767873535, -297.1437322776046130, -345.0633607831865675 ) ) ;
#58117=CARTESIAN_POINT ( 'NONE',  ( -108.8390751952717324, -279.7026395955065823, -254.4438492254772370 ) ) ;
#58118=CARTESIAN_POINT ( 'NONE',  ( 22.69367743960799899, -290.1692442227603124, -315.5914382344669775 ) ) ;
#58121=CARTESIAN_POINT ( 'NONE',  ( 37.80765212740534764, -295.5787231040843039, -278.7109828355824561 ) ) ;
#58122=CARTESIAN_POINT ( 'NONE',  ( -96.03366072200009285, -275.9099979583385789, -317.0748345797995853 ) ) ;
#58123=CARTESIAN_POINT ( 'NONE',  ( -81.82855832738623292, -290.6601124348729854, -207.7106729114560437 ) ) ;
#58124=CARTESIAN_POINT ( 'NONE',  ( 36.09351406484742597, -291.8499248358819500, -262.5371335739541792 ) ) ;
#58125=CARTESIAN_POINT ( 'NONE',  ( -108.4454746125458939, -277.4813229767582357, -251.7241876869527175 ) ) ;
#58126=CARTESIAN_POINT ( 'NONE',  ( -111.6203922558816828, -294.6774983837302671, -271.4581198762632539 ) ) ;
#58127=CARTESIAN_POINT ( 'NONE',  ( -66.77686560023559537, -292.9733686963554078, -203.0200865626528923 ) ) ;
#58128=CARTESIAN_POINT ( 'NONE',  ( 21.27581636871892101, -277.4090924074130839, -223.5744983911110353 ) ) ;
#58129=CARTESIAN_POINT ( 'NONE',  ( -94.14848543269195602, -294.3343536260022120, -321.3285737856231208 ) ) ;
#58130=CARTESIAN_POINT ( 'NONE',  ( -39.96620742770257806, -290.6856771952818690, -344.1645583920227978 ) ) ;
#58131=CARTESIAN_POINT ( 'NONE',  ( -96.65829578305333314, -289.4366997935707104, -222.8688502139236221 ) ) ;
#58132=CARTESIAN_POINT ( 'NONE',  ( -66.54630436392351100, -290.8674575965489453, -337.9615916549828967 ) ) ;
#58134=CARTESIAN_POINT ( 'NONE',  ( -53.43411977051503925, -290.0667442679009582, -341.7308297408944782 ) ) ;
#58136=CARTESIAN_POINT ( 'NONE',  ( 30.02086805183671459, -289.2327344315385176, -306.9452775134249123 ) ) ;
#58137=CARTESIAN_POINT ( 'NONE',  ( -94.63840741837749704, -277.2470690740486248, -221.3975218768623563 ) ) ;
#58138=CARTESIAN_POINT ( 'NONE',  ( -86.79438808761707946, -279.7195724562905639, -211.2986212505088588 ) ) ;
#58139=CARTESIAN_POINT ( 'NONE',  ( 38.40400318723140316, -281.3914658198540906, -284.1577490257680552 ) ) ;
#58140=CARTESIAN_POINT ( 'NONE',  ( 5.898681362571513098, -284.6378285777316819, -209.0172929725891890 ) ) ;
#58142=CARTESIAN_POINT ( 'NONE',  ( 36.93846939916910088, -279.7046024831439581, -271.3535212377353787 ) ) ;
#58143=CARTESIAN_POINT ( 'NONE',  ( -51.76309827054496537, -283.8676133526888634, -196.7077099370488042 ) ) ;
#58145=CARTESIAN_POINT ( 'NONE',  ( -113.6914920201685675, -277.0166758763592156, -271.5778457032989763 ) ) ;
#58147=CARTESIAN_POINT ( 'NONE',  ( -114.0461692048122728, -283.4415372073010531, -272.8255267826199884 ) ) ;
#58148=CARTESIAN_POINT ( 'NONE',  ( -106.4622846741645219, -273.6731683360382021, -246.3830755511384325 ) ) ;
#58149=CARTESIAN_POINT ( 'NONE',  ( -111.0458907210802693, -292.2130409872805217, -265.7052345044734807 ) ) ;
#58150=CARTESIAN_POINT ( 'NONE',  ( -113.7524713807139705, -273.9771950811366992, -270.3792247829380813 ) ) ;
#58151=CARTESIAN_POINT ( 'NONE',  ( -13.78259093020018966, -276.4046617866653150, -339.5305187275776575 ) ) ;
#58152=CARTESIAN_POINT ( 'NONE',  ( -4.647247290047434198, -296.6216490848483431, -337.8740016912877309 ) ) ;
#58153=CARTESIAN_POINT ( 'NONE',  ( -41.75843606997117519, -289.2729999745291138, -347.2475633928224283 ) ) ;
#58154=CARTESIAN_POINT ( 'NONE',  ( 37.24242959245018625, -279.7872982877071308, -282.5463993290489952 ) ) ;
#58156=CARTESIAN_POINT ( 'NONE',  ( 21.31182469501179710, -292.7126773535778170, -220.4534602408569981 ) ) ;
#58157=CARTESIAN_POINT ( 'NONE',  ( -75.09064724807500113, -290.5949536241686815, -207.5450421195383512 ) ) ;
#58158=CARTESIAN_POINT ( 'NONE',  ( 23.25493510020844568, -292.1544723400600674, -314.5760494118696897 ) ) ;
#58162=CARTESIAN_POINT ( 'NONE',  ( -95.15924850839601845, -290.6881560999083263, -225.6943569499026694 ) ) ;
#58164=CARTESIAN_POINT ( 'NONE',  ( -87.60495630512930632, -286.3119319893715442, -212.2698325297329518 ) ) ;
#58165=CARTESIAN_POINT ( 'NONE',  ( -102.0455923789670294, -299.4805209788416391, -239.2376011013261916 ) ) ;
#58166=CARTESIAN_POINT ( 'NONE',  ( 8.755272314045448923, -293.4960405479972678, -331.7442536467502805 ) ) ;
#58167=CARTESIAN_POINT ( 'NONE',  ( -97.64531095546610118, -285.2341442602851203, -317.4437346898933470 ) ) ;
#58168=CARTESIAN_POINT ( 'NONE',  ( -91.51979591788378343, -285.0868590290985480, -221.3610445873512163 ) ) ;
#58169=CARTESIAN_POINT ( 'NONE',  ( 21.40120753946386856, -277.6916707330460667, -314.8580679110328333 ) ) ;
#58170=CARTESIAN_POINT ( 'NONE',  ( 19.20224966008033007, -292.2512021112938214, -319.1107590957861930 ) ) ;
#58171=CARTESIAN_POINT ( 'NONE',  ( -2.649204134466999871, -296.3469020013373552, -335.7400498873485049 ) ) ;
#58174=CARTESIAN_POINT ( 'NONE',  ( 35.99787384989392081, -274.3993974097767818, -274.3494230838704766 ) ) ;
#58177=CARTESIAN_POINT ( 'NONE',  ( -27.75467754098094630, -294.6004269303717251, -346.7939301232727871 ) ) ;
#58178=CARTESIAN_POINT ( 'NONE',  ( 36.98896478362897255, -289.4090146425779153, -265.4681568108989609 ) ) ;
#58179=CARTESIAN_POINT ( 'NONE',  ( 201.0756561822067283, 294.6070805894804039, -54.00000000001602984 ) ) ;
#58180=CARTESIAN_POINT ( 'NONE',  ( -108.6064754957646414, -297.9942967510186804, -241.8841888743917252 ) ) ;
#58181=CARTESIAN_POINT ( 'NONE',  ( -37.28911722089344494, -286.7042057330593821, -197.2467474533602001 ) ) ;
#58182=CARTESIAN_POINT ( 'NONE',  ( -114.1496692561285897, -277.5954527040032644, -271.5926221306101525 ) ) ;
#58183=CARTESIAN_POINT ( 'NONE',  ( -2.006923001309273147, -295.2480227849424068, -338.6602125031901664 ) ) ;
#58184=CARTESIAN_POINT ( 'NONE',  ( 0.08811404618136316202, -286.6994295562074058, -336.2938687728841956 ) ) ;
#58185=CARTESIAN_POINT ( 'NONE',  ( -109.4162445723863613, -296.5416390757753788, -297.5485770366490215 ) ) ;
#58186=CARTESIAN_POINT ( 'NONE',  ( -9.723414220745366876, -292.7562889745286157, -202.7105900535066496 ) ) ;
#58188=CARTESIAN_POINT ( 'NONE',  ( 199.3125048137908948, 285.7142621462966758, -96.33704470926366525 ) ) ;
#58189=CARTESIAN_POINT ( 'NONE',  ( -12.94387731139556230, -287.8837015179771015, -198.0599838732290152 ) ) ;
#58190=CARTESIAN_POINT ( 'NONE',  ( 13.79469577742117181, -291.9094976428775681, -334.5364918783848793 ) ) ;
#58191=VERTEX_POINT ( 'NONE', #23407 ) ;
#58192=CARTESIAN_POINT ( 'NONE',  ( -112.6160518909101143, -278.0983804025460699, -254.5787211769742271 ) ) ;
#58193=CARTESIAN_POINT ( 'NONE',  ( -64.70254933119690577, -285.4104154456896936, -340.0131987695918383 ) ) ;
#58194=CARTESIAN_POINT ( 'NONE',  ( -57.58224511544654689, -284.3706881286718726, -196.6249433411143741 ) ) ;
#58195=CARTESIAN_POINT ( 'NONE',  ( -31.78785177576666499, -287.0615003758479133, -344.6452725989614692 ) ) ;
#58196=CARTESIAN_POINT ( 'NONE',  ( 37.50363879299571579, -277.2619328982166280, -258.5098731277219599 ) ) ;
#58197=CARTESIAN_POINT ( 'NONE',  ( -109.2015176975791348, -296.8696473118008612, -283.6271734132493521 ) ) ;
#58199=CARTESIAN_POINT ( 'NONE',  ( -6.573601784386866598, -293.3242419362358078, -337.1036651603427572 ) ) ;
#58200=CARTESIAN_POINT ( 'NONE',  ( -90.99300181464917614, -279.9661299703982422, -215.1973980773842641 ) ) ;
#58201=CARTESIAN_POINT ( 'NONE',  ( -71.65418411124608156, -277.5188250187982248, -334.8085431949305644 ) ) ;
#58202=CARTESIAN_POINT ( 'NONE',  ( -106.5385291618271282, -278.2154274947003501, -246.6326131620838851 ) ) ;
#58203=CARTESIAN_POINT ( 'NONE',  ( -29.88268093593819330, -275.2241496302303858, -194.0338257326666564 ) ) ;
#58204=CARTESIAN_POINT ( 'NONE',  ( -31.48763716215004393, -275.9003400867459845, -346.8806632889305774 ) ) ;
#58205=CARTESIAN_POINT ( 'NONE',  ( 43.54794645580765433, 12.48440977809399044, -329.5723226709832261 ) ) ;
#58206=CARTESIAN_POINT ( 'NONE',  ( -113.7489416061644079, -297.9866821896073930, -269.6264473118700948 ) ) ;
#58207=CARTESIAN_POINT ( 'NONE',  ( -4.771743288812468897, -279.1233781216988064, -337.9199732462171255 ) ) ;
#58209=CARTESIAN_POINT ( 'NONE',  ( -65.22346980029674057, -286.7588089258796913, -202.5071288061722896 ) ) ;
#58210=CARTESIAN_POINT ( 'NONE',  ( -37.99650225805415715, -287.8041885670105557, -194.3772693592969745 ) ) ;
#58211=CARTESIAN_POINT ( 'NONE',  ( -13.26211249848714324, -288.0795226656879322, -339.3833327229949646 ) ) ;
#58212=CARTESIAN_POINT ( 'NONE',  ( -108.5979489720030386, -276.7010437375448078, -289.5701631780463003 ) ) ;
#58213=CARTESIAN_POINT ( 'NONE',  ( -99.14837876029218933, -286.9738533148823194, -229.2417799922106951 ) ) ;
#58214=CARTESIAN_POINT ( 'NONE',  ( -105.0717616871353641, -277.4184846410717000, -241.3206890615510076 ) ) ;
#58216=CARTESIAN_POINT ( 'NONE',  ( 1.143847806879024098, -277.8422096930956400, -333.0316737654466124 ) ) ;
#58217=CARTESIAN_POINT ( 'NONE',  ( -1.698082109681582796, -275.0304308408280463, -206.5696738322164947 ) ) ;
#58218=CARTESIAN_POINT ( 'NONE',  ( 37.71613785676404262, -286.5395197339906304, -285.6689485586093156 ) ) ;
#58219=CARTESIAN_POINT ( 'NONE',  ( 39.36866596328303558, -282.4211365566412155, -275.6395980569988637 ) ) ;
#58220=CARTESIAN_POINT ( 'NONE',  ( 17.78656414352937531, -282.7815930854620774, -324.1066213702296750 ) ) ;
#58224=CARTESIAN_POINT ( 'NONE',  ( -40.26696085343008491, -290.9489359918557625, -346.0823009421269489 ) ) ;
#58225=CARTESIAN_POINT ( 'NONE',  ( -89.16978683164447261, -288.4482152006335127, -326.6385353037309187 ) ) ;
#58226=CARTESIAN_POINT ( 'NONE',  ( -74.20133298768131169, -297.1333645920589106, -337.1120908320992839 ) ) ;
#58228=CARTESIAN_POINT ( 'NONE',  ( -51.59555791091181476, -272.9242197864306263, -198.4743806370645416 ) ) ;
#58229=CARTESIAN_POINT ( 'NONE',  ( 19.34613559413926609, -292.1929228355894566, -218.4014983941503658 ) ) ;
#58230=CARTESIAN_POINT ( 'NONE',  ( 20.04129323010142016, -286.6796297856447495, -316.5985468466306543 ) ) ;
#58231=CARTESIAN_POINT ( 'NONE',  ( -37.53033859561809749, -290.2896533367708116, -196.3354047945619243 ) ) ;
#58232=CARTESIAN_POINT ( 'NONE',  ( 33.04642829373552360, -288.4829575368902965, -249.5167688308048071 ) ) ;
#58233=CARTESIAN_POINT ( 'NONE',  ( -20.25526795762937127, -288.7662352645560304, -195.3538533559490702 ) ) ;
#58234=CARTESIAN_POINT ( 'NONE',  ( 2.149281404534636231, -290.5239512994888287, -334.1830368055075837 ) ) ;
#58235=CARTESIAN_POINT ( 'NONE',  ( -107.7474599451786474, -288.8947816879293669, -243.8869396391374949 ) ) ;
#58236=CARTESIAN_POINT ( 'NONE',  ( -73.06487903641890114, -293.5788905872786358, -204.4008426570613324 ) ) ;
#58237=CARTESIAN_POINT ( 'NONE',  ( -108.8973677438136463, -285.6992358728543877, -254.7078203641029575 ) ) ;
#58238=CARTESIAN_POINT ( 'NONE',  ( 37.61099674567384454, -295.4797054373212291, -264.6935209884815663 ) ) ;
#58241=CARTESIAN_POINT ( 'NONE',  ( -94.79046025150023524, -275.2039058364813968, -221.5760213046299327 ) ) ;
#58243=CARTESIAN_POINT ( 'NONE',  ( 3.471842861263185309, -281.6852602607441440, -331.1418827868079120 ) ) ;
#58244=CARTESIAN_POINT ( 'NONE',  ( -48.65483276734726559, -281.1960574157956785, -344.5029663300841776 ) ) ;
#58245=CARTESIAN_POINT ( 'NONE',  ( -111.0633602407238669, -295.4764985487591389, -292.0703197071943578 ) ) ;
#58246=CARTESIAN_POINT ( 'NONE',  ( -1.208604281813214998, -272.7783061427584812, -205.7526923375826868 ) ) ;
#58247=CARTESIAN_POINT ( 'NONE',  ( -83.92659682963245871, -275.7771677919594708, -328.4891815762184706 ) ) ;
#58248=CARTESIAN_POINT ( 'NONE',  ( -108.3162505107594740, -298.1181574629493412, -251.2375541694671313 ) ) ;
#58249=CARTESIAN_POINT ( 'NONE',  ( -111.3244174429133153, -294.5716042925540705, -287.7533129690814917 ) ) ;
#58250=CARTESIAN_POINT ( 'NONE',  ( -34.25848560582333846, -296.4379044670329790, -343.8857309122151378 ) ) ;
#58253=CARTESIAN_POINT ( 'NONE',  ( -82.45135474656788688, -296.4888317288817916, -328.0253619373830247 ) ) ;
#58255=CARTESIAN_POINT ( 'NONE',  ( -46.28474187098094461, -283.9593236050528162, -195.5384689663494555 ) ) ;
#58256=CARTESIAN_POINT ( 'NONE',  ( -86.48997559454481632, -295.7579594095685138, -324.3374740903284419 ) ) ;
#58257=CARTESIAN_POINT ( 'NONE',  ( -85.51291023190965745, -285.4066929034167970, -210.2900391081729197 ) ) ;
#58258=CARTESIAN_POINT ( 'NONE',  ( 20.52330978778046244, -284.1389681587759810, -318.9507756119650139 ) ) ;
#58259=CARTESIAN_POINT ( 'NONE',  ( 37.69997151749419118, -287.0035354326991524, -253.1418385239699944 ) ) ;
#58260=CARTESIAN_POINT ( 'NONE',  ( -37.52961080354226908, -290.0496729250559724, -195.5152595537584261 ) ) ;
#58261=CARTESIAN_POINT ( 'NONE',  ( -79.81299671697057363, -278.6911714272116001, -206.2633394766397146 ) ) ;
#58262=CARTESIAN_POINT ( 'NONE',  ( -4.829096099716524648, -274.1237833571632905, -337.9475929042657754 ) ) ;
#58264=CARTESIAN_POINT ( 'NONE',  ( 27.37336643614064258, -286.8178523263323427, -305.0971347635345978 ) ) ;
#58265=CARTESIAN_POINT ( 'NONE',  ( -112.3347911955533220, -289.6747346766688906, -254.2515097302040488 ) ) ;
#58267=LINE ( 'NONE', #8039, #47570 ) ;
#58268=CARTESIAN_POINT ( 'NONE',  ( -99.39504528137669581, -297.6042929491894711, -310.4024476261736822 ) ) ;
#58269=CARTESIAN_POINT ( 'NONE',  ( 16.79275225609071143, -282.2293584035601270, -216.3604446281086382 ) ) ;
#58270=CARTESIAN_POINT ( 'NONE',  ( -93.44423988109707579, -293.8746576548170992, -320.6885192881327953 ) ) ;
#58271=CARTESIAN_POINT ( 'NONE',  ( 25.15658005934236741, -280.6980527056792880, -232.5000114213190443 ) ) ;
#58272=CARTESIAN_POINT ( 'NONE',  ( -64.26419870252848909, -295.5606178369052941, -342.5011143438870249 ) ) ;
#58273=CARTESIAN_POINT ( 'NONE',  ( -1.628175471129533314, -284.6016003994726589, -203.7738943087226744 ) ) ;
#58274=CARTESIAN_POINT ( 'NONE',  ( -111.2694996848005076, -280.7145634904664462, -257.7246191395745996 ) ) ;
#58275=CARTESIAN_POINT ( 'NONE',  ( -88.28082168808782626, -296.3763200922820715, -217.6727039389922425 ) ) ;
#58277=CARTESIAN_POINT ( 'NONE',  ( -23.74162510921650338, -284.8574079056663777, -343.7565181063085902 ) ) ;
#58279=CARTESIAN_POINT ( 'NONE',  ( -54.42813229853333468, -289.3380690714489560, -195.3538533559490702 ) ) ;
#58280=CARTESIAN_POINT ( 'NONE',  ( -41.17446446268515814, -273.2023711190662425, -193.5660932937568361 ) ) ;
#58281=CARTESIAN_POINT ( 'NONE',  ( -77.25338171711713642, -291.3337096023544177, -209.2378190104927285 ) ) ;
#58282=CARTESIAN_POINT ( 'NONE',  ( 20.20541809279164269, -282.4280167481900889, -224.3281196089028242 ) ) ;
#58283=CARTESIAN_POINT ( 'NONE',  ( 5.626158736696218909, -276.2448270859183026, -210.2962727238852096 ) ) ;
#58284=CARTESIAN_POINT ( 'NONE',  ( 35.71756369356082672, -283.4288389259120891, -292.1942368075359013 ) ) ;
#58285=CARTESIAN_POINT ( 'NONE',  ( 36.08497729768387075, -280.3238216147161097, -268.5892202236719299 ) ) ;
#58286=CARTESIAN_POINT ( 'NONE',  ( -112.3522940074298333, -280.5843480021209189, -267.8664730575142698 ) ) ;
#58287=CARTESIAN_POINT ( 'NONE',  ( -14.81011945751415482, -298.3269540641308026, -193.3611147766884812 ) ) ;
#58288=CARTESIAN_POINT ( 'NONE',  ( -1.299615256720735079, -274.3501664142771688, -202.3172488785206440 ) ) ;
#58289=CARTESIAN_POINT ( 'NONE',  ( 37.14909936406689184, -295.4772581778345852, -270.7433852963139884 ) ) ;
#58292=CARTESIAN_POINT ( 'NONE',  ( 29.79665691587037912, -292.1521233984457240, -305.4716077447148450 ) ) ;
#58293=CARTESIAN_POINT ( 'NONE',  ( -65.83136517139847399, -273.1767455329260770, -203.0831317798035798 ) ) ;
#58294=CARTESIAN_POINT ( 'NONE',  ( -16.83174482472171718, -293.8325048609812029, -196.8624820461997160 ) ) ;
#58295=CARTESIAN_POINT ( 'NONE',  ( -69.91165696735023971, -282.1233781216988064, -202.8022627189028810 ) ) ;
#58296=CARTESIAN_POINT ( 'NONE',  ( 27.70702231335044274, -294.2241103729919018, -229.8051125037101770 ) ) ;
#58297=CARTESIAN_POINT ( 'NONE',  ( -59.20092442257989518, -291.3357502869835116, -341.9848071854732439 ) ) ;
#58298=CARTESIAN_POINT ( 'NONE',  ( -105.0172135804407532, -276.9744033416577054, -238.3011358862991074 ) ) ;
#58299=CARTESIAN_POINT ( 'NONE',  ( -18.63185683874331389, -278.7294627613449620, -342.4114889677319411 ) ) ;
#58300=CARTESIAN_POINT ( 'NONE',  ( 30.79856729035514817, -292.0274114234154581, -300.3314057892122833 ) ) ;
#58301=CARTESIAN_POINT ( 'NONE',  ( 18.88305533748748033, -284.1140494761307878, -321.2225697128147317 ) ) ;
#58304=CARTESIAN_POINT ( 'NONE',  ( -61.54573377576387827, -283.0420229885423282, -339.3074201879663860 ) ) ;
#58305=CARTESIAN_POINT ( 'NONE',  ( -1.292939957813983964, -281.5986279731169475, -202.6707981383232777 ) ) ;
#58306=CARTESIAN_POINT ( 'NONE',  ( -37.32979979347020105, -281.8469005615052083, -346.9770435935736259 ) ) ;
#58307=CARTESIAN_POINT ( 'NONE',  ( -38.52926204500557361, -278.0079491449293414, -347.1166383744142649 ) ) ;
#58309=CARTESIAN_POINT ( 'NONE',  ( 0.7181685609744621335, -278.0747575706834027, -336.5584474768193672 ) ) ;
#58310=CARTESIAN_POINT ( 'NONE',  ( -105.5937364680635966, -287.2662352645559167, -254.8156830097664738 ) ) ;
#58311=ORIENTED_EDGE ( 'NONE', *, *, #51345, .F. ) ;
#58312=CARTESIAN_POINT ( 'NONE',  ( -96.03189373401131945, -299.1941044660121634, -223.6657024873655928 ) ) ;
#58313=CARTESIAN_POINT ( 'NONE',  ( -104.6242799427030974, -276.1431822857979910, -302.8057335621401194 ) ) ;
#58314=CARTESIAN_POINT ( 'NONE',  ( -113.0001561734949718, -292.4086110728650283, -262.7608981482744639 ) ) ;
#58315=CARTESIAN_POINT ( 'NONE',  ( 32.44163992935142460, -293.1888975920410871, -292.1367492862830773 ) ) ;
#58316=CARTESIAN_POINT ( 'NONE',  ( -23.32930461582569137, -288.3853854432213666, -346.0668884496899409 ) ) ;
#58318=CARTESIAN_POINT ( 'NONE',  ( -33.48288683644734931, -293.5792349356514706, -346.6874115249253805 ) ) ;
#58319=CARTESIAN_POINT ( 'NONE',  ( -103.7412543665334965, -282.5193067332134547, -302.6894106360171577 ) ) ;
#58320=CARTESIAN_POINT ( 'NONE',  ( -53.65733380765710336, -291.1241574246280379, -342.7811813286864435 ) ) ;
#58321=CARTESIAN_POINT ( 'NONE',  ( -84.07272947292911169, -283.8765298433623343, -213.3130897672952528 ) ) ;
#58323=CARTESIAN_POINT ( 'NONE',  ( 20.57991198015645651, -283.5006407618025719, -315.5975007996236172 ) ) ;
#58324=CARTESIAN_POINT ( 'NONE',  ( -114.0157034834198413, -291.4466031181196399, -274.0917240732396181 ) ) ;
#58325=CARTESIAN_POINT ( 'NONE',  ( 17.10448985719286341, -281.3480500589778899, -221.6415034741993679 ) ) ;
#58326=CARTESIAN_POINT ( 'NONE',  ( 27.76032930563117418, -292.8789244679813919, -310.8307130154411766 ) ) ;
#58327=CARTESIAN_POINT ( 'NONE',  ( -51.64520337528083616, -290.0334952358699070, -345.8566053634414743 ) ) ;
#58328=CARTESIAN_POINT ( 'NONE',  ( 39.28671753018082313, -288.1308634148895749, -277.2612998862767313 ) ) ;
#58329=CARTESIAN_POINT ( 'NONE',  ( -22.46190960699132333, -286.4145475870277551, -198.8418196244562068 ) ) ;
#58332=CARTESIAN_POINT ( 'NONE',  ( -2.513844428382396412, -296.4568300006881145, -337.6465246511868372 ) ) ;
#58333=CARTESIAN_POINT ( 'NONE',  ( -90.38233155883600034, -294.4685323130469214, -325.5701738207189919 ) ) ;
#58335=CARTESIAN_POINT ( 'NONE',  ( -108.1971956605758862, -277.8551845426517275, -251.7941372455289013 ) ) ;
#58336=CARTESIAN_POINT ( 'NONE',  ( -93.12322679337654563, -272.7847640493824883, -217.3518174516033525 ) ) ;
#58337=CARTESIAN_POINT ( 'NONE',  ( 1.923027429044345871, -292.9965976159466550, -332.7833032779283826 ) ) ;
#58338=CARTESIAN_POINT ( 'NONE',  ( 21.47332155501657525, -276.6888042994611965, -225.4095706447155010 ) ) ;
#58339=CARTESIAN_POINT ( 'NONE',  ( -111.4196221396391309, -270.7638995432500337, -264.7976786683124146 ) ) ;
#58340=CARTESIAN_POINT ( 'NONE',  ( 35.93001590074437246, -294.6904849177667529, -265.2736132104790840 ) ) ;
#58341=CARTESIAN_POINT ( 'NONE',  ( 35.92984866486841611, -294.6010057665943123, -268.0145864630187020 ) ) ;
#58343=CARTESIAN_POINT ( 'NONE',  ( -103.6246451176777015, -295.0225600455010522, -234.8022235856830093 ) ) ;
#58344=CARTESIAN_POINT ( 'NONE',  ( -33.34939872976709552, -298.7523158506616596, -193.4626218776420785 ) ) ;
#58346=CARTESIAN_POINT ( 'NONE',  ( -45.37639676859437543, -290.0977039935931430, -343.1543326239825547 ) ) ;
#58347=CARTESIAN_POINT ( 'NONE',  ( -86.50107905408648890, -296.0911869259354603, -324.3559598687174343 ) ) ;
#58348=CARTESIAN_POINT ( 'NONE',  ( -110.8040164433576535, -280.7465249094090609, -253.5773493502111364 ) ) ;
#58349=CARTESIAN_POINT ( 'NONE',  ( -112.5837081757703686, -277.0616934021779798, -284.2873674300295193 ) ) ;
#58351=CARTESIAN_POINT ( 'NONE',  ( -2.945886374331133428, -281.9582400045186432, -339.1524971229500807 ) ) ;
#58352=CARTESIAN_POINT ( 'NONE',  ( 39.03533141284781038, -275.0182385929391558, -279.7437039210689704 ) ) ;
#58353=CARTESIAN_POINT ( 'NONE',  ( -38.94004221035388014, -281.1521692368178265, -344.7966975744905653 ) ) ;
#58354=CARTESIAN_POINT ( 'NONE',  ( -97.05712984982912417, -277.5921178540615983, -223.0271146448996546 ) ) ;
#58355=CARTESIAN_POINT ( 'NONE',  ( 22.30836163735874322, -278.9268243332195425, -224.6028050068051982 ) ) ;
#58356=CARTESIAN_POINT ( 'NONE',  ( -77.76937007875561392, -296.1818657568402386, -208.9253288462895739 ) ) ;
#58357=CARTESIAN_POINT ( 'NONE',  ( 2.934614965450828894, -276.5925159262648663, -207.0330154259141864 ) ) ;
#58359=CARTESIAN_POINT ( 'NONE',  ( -33.59536954915453322, -290.1192024457285470, -195.0990969376645126 ) ) ;
#58360=CARTESIAN_POINT ( 'NONE',  ( -46.02577120096609775, -289.1592547759493073, -346.9229821982838757 ) ) ;
#58361=CARTESIAN_POINT ( 'NONE',  ( -69.37420419624034196, -275.6318797648829673, -202.3474349208476326 ) ) ;
#58362=CARTESIAN_POINT ( 'NONE',  ( -37.80903230386057601, -296.0461271034363904, -195.5292395371845089 ) ) ;
#58363=CARTESIAN_POINT ( 'NONE',  ( -112.0645266158754509, -283.5242046485086007, -288.3237726859858299 ) ) ;
#58365=CARTESIAN_POINT ( 'NONE',  ( -73.13966234031319402, -283.5774948242063829, -204.4414870264439230 ) ) ;
#58366=CARTESIAN_POINT ( 'NONE',  ( -41.60061644141435266, -290.7923801535328039, -197.0375931494471047 ) ) ;
#58367=CARTESIAN_POINT ( 'NONE',  ( -96.74027365681310187, -283.3063994716749221, -225.8338797403751528 ) ) ;
#58369=CARTESIAN_POINT ( 'NONE',  ( 33.70357676229919264, -291.2393223269993996, -246.1666149264316630 ) ) ;
#58370=CARTESIAN_POINT ( 'NONE',  ( -106.3865933676369337, -282.6121198319348764, -302.8497385815358030 ) ) ;
#58371=CARTESIAN_POINT ( 'NONE',  ( -51.41368808682262426, -278.8352365515879683, -342.8070948757865608 ) ) ;
#58372=CARTESIAN_POINT ( 'NONE',  ( -91.63244968300998039, -286.5043490144807947, -216.3192524442690114 ) ) ;
#58373=CARTESIAN_POINT ( 'NONE',  ( -108.3655117301545090, -284.7753603036408094, -253.4366518807889577 ) ) ;
#58374=CARTESIAN_POINT ( 'NONE',  ( -24.20674488962405135, -278.3065669367290411, -342.8204983278910731 ) ) ;
#58375=CARTESIAN_POINT ( 'NONE',  ( -110.0633499866582099, -279.2436668163700233, -278.8186138284518165 ) ) ;
#58376=CARTESIAN_POINT ( 'NONE',  ( -68.97316281992121390, -287.6364293412214579, -202.3438063100544184 ) ) ;
#58378=CARTESIAN_POINT ( 'NONE',  ( -103.1166882382116228, -295.8627293820108548, -310.3942410634140288 ) ) ;
#58379=CARTESIAN_POINT ( 'NONE',  ( 24.11818541854335152, -290.1092448805503068, -312.7455431087248030 ) ) ;
#58381=CARTESIAN_POINT ( 'NONE',  ( -37.30987171927208124, -279.5519495502701375, -350.3611179825600175 ) ) ;
#58382=CARTESIAN_POINT ( 'NONE',  ( -111.5319239254870638, -277.2277796176067000, -289.8370487943196849 ) ) ;
#58383=CARTESIAN_POINT ( 'NONE',  ( 28.79154415393354327, -291.4550830934755936, -232.5083186862884759 ) ) ;
#58385=CARTESIAN_POINT ( 'NONE',  ( 0.5083090456454590900, -288.0861827630913012, -207.0712265881521716 ) ) ;
#58386=CARTESIAN_POINT ( 'NONE',  ( -108.9587208051619172, -280.5561409695507677, -251.6303671650568106 ) ) ;
#58387=CARTESIAN_POINT ( 'NONE',  ( 21.62380842631358036, -288.3194165706153740, -221.7640491826302309 ) ) ;
#58388=CARTESIAN_POINT ( 'NONE',  ( -81.79152836529674175, -285.6572679374419863, -330.8344369047159148 ) ) ;
#58389=CARTESIAN_POINT ( 'NONE',  ( -100.4642887699044422, -278.1359051998626342, -314.4580431323665266 ) ) ;
#58390=CARTESIAN_POINT ( 'NONE',  ( -108.0300300901720476, -270.8706271181288230, -245.8012231799324638 ) ) ;
#58391=CARTESIAN_POINT ( 'NONE',  ( 35.69705332690548261, -291.3844836661102136, -250.9551376928707498 ) ) ;
#58392=CARTESIAN_POINT ( 'NONE',  ( -36.75042222319528662, -279.8927125155788644, -193.3503426217190793 ) ) ;
#58393=CARTESIAN_POINT ( 'NONE',  ( -97.29268955086435255, -275.0163984807197153, -226.4950400131153572 ) ) ;
#58395=CARTESIAN_POINT ( 'NONE',  ( -106.6379572354042296, -286.6233781216988064, -303.7686719486574702 ) ) ;
#58396=CARTESIAN_POINT ( 'NONE',  ( -82.95368798358974516, -271.6779514111104277, -209.5209363602475037 ) ) ;
#58398=CARTESIAN_POINT ( 'NONE',  ( -19.51347483645707825, -279.7952200927817330, -199.4558163882677206 ) ) ;
#58399=CARTESIAN_POINT ( 'NONE',  ( 30.20024625159727094, -277.2279935711843564, -306.6130853767727444 ) ) ;
#58400=CARTESIAN_POINT ( 'NONE',  ( -40.56177513122295153, -299.4361782809191936, -196.8297219094943955 ) ) ;
#58401=CARTESIAN_POINT ( 'NONE',  ( -110.4650802941433625, -283.3157995425652302, -293.7666687723445875 ) ) ;
#58402=CARTESIAN_POINT ( 'NONE',  ( 4.201671596619388716, -290.2442596623231452, -331.6774983679813431 ) ) ;
#58403=CARTESIAN_POINT ( 'NONE',  ( -80.25128087289158429, -299.0030292917705310, -207.1986425440775861 ) ) ;
#58404=CARTESIAN_POINT ( 'NONE',  ( -65.41087712666603693, -298.8984625365128522, -199.0293866496947999 ) ) ;
#58405=CARTESIAN_POINT ( 'NONE',  ( 28.78986439202218861, -296.0189989776899893, -305.4954043938395216 ) ) ;
#58406=CARTESIAN_POINT ( 'NONE',  ( -18.29294820875840344, -280.8060991768934400, -342.7831508123792901 ) ) ;
#58407=CARTESIAN_POINT ( 'NONE',  ( -106.9409264893640739, -270.9264703521370734, -243.2409976749496536 ) ) ;
#58408=CARTESIAN_POINT ( 'NONE',  ( -68.19570451451193094, -287.2538163752089986, -200.6728563515134738 ) ) ;
#58409=CARTESIAN_POINT ( 'NONE',  ( 22.99653746753078210, -287.0501751632339165, -312.0188389156088533 ) ) ;
#58410=CARTESIAN_POINT ( 'NONE',  ( 191.0571775945797413, 270.4395961937442507, -139.4957094208748742 ) ) ;
#58412=CARTESIAN_POINT ( 'NONE',  ( -77.83962550829022575, -288.1591423404382226, -335.2188682935441193 ) ) ;
#58413=CARTESIAN_POINT ( 'NONE',  ( -50.75951370256545658, -288.8948812734350895, -342.1905927832334555 ) ) ;
#58415=CARTESIAN_POINT ( 'NONE',  ( -52.12721194931695834, -286.9469496106779047, -195.0548270488407354 ) ) ;
#58416=CARTESIAN_POINT ( 'NONE',  ( 7.596744947866507225, -276.7530111416994032, -327.9809476184909727 ) ) ;
#58417=CARTESIAN_POINT ( 'NONE',  ( 26.24772262053544125, -293.0396140204292124, -313.2315952860676020 ) ) ;
#58418=CARTESIAN_POINT ( 'NONE',  ( -94.31804429160564496, -284.5008879551541554, -322.0237375709436947 ) ) ;
#58420=CARTESIAN_POINT ( 'NONE',  ( 14.67442708935393547, -282.2884918934940970, -214.4585334762561502 ) ) ;
#58421=CARTESIAN_POINT ( 'NONE',  ( -27.37063287721139915, -283.2621669158975806, -346.7448132276550155 ) ) ;
#58422=CARTESIAN_POINT ( 'NONE',  ( -7.994842286096558226, -280.7807800616295140, -203.4830312952278746 ) ) ;
#58423=CARTESIAN_POINT ( 'NONE',  ( -47.91463450998808327, -155.0658791552682771, -365.2963413022445138 ) ) ;
#58424=CARTESIAN_POINT ( 'NONE',  ( -41.94452411973847461, -279.1104285115721382, -345.0656798433621475 ) ) ;
#58425=CARTESIAN_POINT ( 'NONE',  ( 172.9411727994402099, 243.4788377357485842, -179.2791985832347450 ) ) ;
#58426=CARTESIAN_POINT ( 'NONE',  ( -63.90417860558302010, -182.1577870710572427, -358.9045216547217478 ) ) ;
#58427=CARTESIAN_POINT ( 'NONE',  ( -63.35460015881222517, -272.9015416359167148, -201.9668177545093783 ) ) ;
#58428=CARTESIAN_POINT ( 'NONE',  ( -64.25054150048123347, -294.9016968972546238, -342.4405266870813875 ) ) ;
#58429=CARTESIAN_POINT ( 'NONE',  ( 161.5460264286427901, 217.5614978313379027, -202.5778412181095121 ) ) ;
#58430=CARTESIAN_POINT ( 'NONE',  ( -95.64096031508621820, -271.9093723775093281, -220.7980970025738543 ) ) ;
#58431=CARTESIAN_POINT ( 'NONE',  ( -73.89024697504872563, -297.4035005713763553, -334.9758934172893419 ) ) ;
#58432=CARTESIAN_POINT ( 'NONE',  ( 35.24893886790719932, -289.0188369879009542, -281.9237046592797356 ) ) ;
#58434=CARTESIAN_POINT ( 'NONE',  ( -16.55902372496308672, -295.7313776441777122, -344.3140911798018351 ) ) ;
#58436=CARTESIAN_POINT ( 'NONE',  ( -52.10749130080926506, -286.3503390200427248, -198.8072232422762227 ) ) ;
#58437=CARTESIAN_POINT ( 'NONE',  ( -99.30912684682645875, -272.0756134916392170, -225.0897810305235680 ) ) ;
#58438=CARTESIAN_POINT ( 'NONE',  ( 35.29660418142283618, -294.0366518311817003, -245.1434749720196464 ) ) ;
#58439=CARTESIAN_POINT ( 'NONE',  ( 39.17656066855866470, -294.1511463385074876, -278.8818188403940894 ) ) ;
#58440=CARTESIAN_POINT ( 'NONE',  ( -94.29224039994291218, -291.3644611793104104, -224.6724901682865720 ) ) ;
#58442=CARTESIAN_POINT ( 'NONE',  ( -32.79416743334270734, -276.0291597398052659, -194.9251785916763424 ) ) ;
#58443=CARTESIAN_POINT ( 'NONE',  ( 25.01266335400542218, -273.7543836994849471, -225.8421324235300744 ) ) ;
#58446=CARTESIAN_POINT ( 'NONE',  ( -97.01064731726852131, -277.4073163381632980, -318.9527672941724745 ) ) ;
#58447=CARTESIAN_POINT ( 'NONE',  ( 36.49894020260426686, -273.9684258395309371, -271.6187131300891906 ) ) ;
#58448=CARTESIAN_POINT ( 'NONE',  ( -102.3107407040983645, -274.0933277833743773, -236.2915980912451346 ) ) ;
#58449=CARTESIAN_POINT ( 'NONE',  ( 29.29517971762503592, -276.0836535979860855, -239.8586449463161046 ) ) ;
#58450=CARTESIAN_POINT ( 'NONE',  ( -67.15893593552482344, -275.4266976211831093, -200.4690121049508775 ) ) ;
#58452=CARTESIAN_POINT ( 'NONE',  ( -23.27128463348706688, -274.8933366422025983, -344.4440705731836943 ) ) ;
#58453=CARTESIAN_POINT ( 'NONE',  ( -109.2408801439398900, -297.0286876214525478, -283.6365004408074242 ) ) ;
#58454=CARTESIAN_POINT ( 'NONE',  ( -10.29015071914576218, -293.2667493695074654, -338.7978668247616270 ) ) ;
#58456=CARTESIAN_POINT ( 'NONE',  ( -25.77302880867310364, -277.4008944307328761, -346.4248593249108126 ) ) ;
#58457=CARTESIAN_POINT ( 'NONE',  ( -5.309972176139226896, -274.6524803298712527, -204.7502788534600029 ) ) ;
#58458=CARTESIAN_POINT ( 'NONE',  ( -113.7172154232418251, -283.1701974516616929, -275.6667871009972828 ) ) ;
#58459=CARTESIAN_POINT ( 'NONE',  ( -103.6486718138149996, -299.0222371873659881, -234.8470467293802812 ) ) ;
#58461=CARTESIAN_POINT ( 'NONE',  ( 13.25860137813144846, -285.9786666956291583, -217.4498359795061617 ) ) ;
#58462=CARTESIAN_POINT ( 'NONE',  ( -105.3646991354110867, -277.1785040204522375, -241.1918598979209207 ) ) ;
#58463=CARTESIAN_POINT ( 'NONE',  ( -106.8265371811337445, -276.8052927607587321, -294.7486472775113953 ) ) ;
#58464=CARTESIAN_POINT ( 'NONE',  ( -96.58657296726110530, -285.9215667679726494, -316.3711900782746511 ) ) ;
#58465=CARTESIAN_POINT ( 'NONE',  ( 13.76218537912401452, -275.9933391362311568, -217.6778816511363743 ) ) ;
#58467=CARTESIAN_POINT ( 'NONE',  ( 20.20258887593741548, -274.6343452175885886, -320.3317878946602377 ) ) ;
#58468=CARTESIAN_POINT ( 'NONE',  ( -89.79745371018157130, -281.3146599572119726, -216.4515332026948897 ) ) ;
#58470=CARTESIAN_POINT ( 'NONE',  ( -4.144497788464432730, -288.4065301653239430, -202.4700646369654748 ) ) ;
#58472=CARTESIAN_POINT ( 'NONE',  ( 13.49681460457306237, -292.3407651114022769, -325.5707990135144883 ) ) ;
#58473=CARTESIAN_POINT ( 'NONE',  ( 82.17345649163328858, -297.6224838372864951, -195.9197544271459606 ) ) ;
#58474=CARTESIAN_POINT ( 'NONE',  ( 95.32732251205690943, -298.5441162442227210, -196.9920762313734599 ) ) ;
#58475=CARTESIAN_POINT ( 'NONE',  ( -110.6424761585032144, -288.5383816393801908, -282.1826822617540529 ) ) ;
#58476=CARTESIAN_POINT ( 'NONE',  ( -72.39245198575343920, -211.1690049852372226, -355.6323962662157783 ) ) ;
#58478=CARTESIAN_POINT ( 'NONE',  ( -111.2553277063197044, -288.7920120299869495, -289.3734906542701424 ) ) ;
#58479=CARTESIAN_POINT ( 'NONE',  ( -40.24565939529109215, -284.6893924604142967, -344.1039646674390724 ) ) ;
#58480=CARTESIAN_POINT ( 'NONE',  ( -68.07015418690684783, -283.8940900190387993, -200.8506301183062703 ) ) ;
#58481=CARTESIAN_POINT ( 'NONE',  ( -59.10521357335203163, -284.7645186904123875, -340.7120839882558130 ) ) ;
#58482=CARTESIAN_POINT ( 'NONE',  ( -109.1359871761006985, -285.1696887219596874, -284.4388335167977289 ) ) ;
#58483=CARTESIAN_POINT ( 'NONE',  ( -37.47286432276283108, -291.0336373613998830, -345.7290011042935589 ) ) ;
#58484=CARTESIAN_POINT ( 'NONE',  ( -36.94410440113354355, -274.3903138879673520, -193.3702402195489469 ) ) ;
#58485=CARTESIAN_POINT ( 'NONE',  ( -29.15790835359109323, -287.0292013679276693, -345.5291511015668107 ) ) ;
#58486=CARTESIAN_POINT ( 'NONE',  ( 39.70739121345921774, -275.5622889030945544, -271.1716430989686160 ) ) ;
#58487=CARTESIAN_POINT ( 'NONE',  ( -9.861535590313803112, -296.6713642364161956, -339.7634764462429189 ) ) ;
#58489=CARTESIAN_POINT ( 'NONE',  ( -20.19161114001083490, -291.3376638359845856, -345.3538533559490702 ) ) ;
#58490=CARTESIAN_POINT ( 'NONE',  ( -69.23824654133224499, -282.1656357340476688, -336.5856934696784606 ) ) ;
#58491=CARTESIAN_POINT ( 'NONE',  ( -73.24414394369171077, -275.5268462595597612, -336.4139582406987188 ) ) ;
#58492=CARTESIAN_POINT ( 'NONE',  ( -95.48669588160079513, -271.7044575634330954, -220.9257532575719551 ) ) ;
#58493=CARTESIAN_POINT ( 'NONE',  ( 0.9177153736660982331, -275.8759394994144145, -332.7111206613425907 ) ) ;
#58494=CARTESIAN_POINT ( 'NONE',  ( 33.28807357263086431, -294.7945328603215103, -249.1582423563963857 ) ) ;
#58495=CARTESIAN_POINT ( 'NONE',  ( 30.06764308909870209, -294.1087670657261128, -241.6064579155074341 ) ) ;
#58496=CARTESIAN_POINT ( 'NONE',  ( -77.61905349252327824, -287.2639421500850858, -208.2059445791758208 ) ) ;
#58497=CARTESIAN_POINT ( 'NONE',  ( -3.598041709504797403, -293.9140065291185806, -201.7903531791220360 ) ) ;
#58498=CARTESIAN_POINT ( 'NONE',  ( 35.81051696178221277, -294.5841558577627097, -247.9546142900702250 ) ) ;
#58499=CARTESIAN_POINT ( 'NONE',  ( -110.3742152570091548, -296.4069778958614165, -268.7307783224857758 ) ) ;
#58500=CARTESIAN_POINT ( 'NONE',  ( -37.24043142775248327, -291.0510410168107569, -345.3610539718976042 ) ) ;
#58501=CARTESIAN_POINT ( 'NONE',  ( -8.036919884285145699, -282.8455554193877788, -341.6232045902410732 ) ) ;
#58502=CARTESIAN_POINT ( 'NONE',  ( -38.31735470500477447, -272.1796342736362817, -194.6025964660167631 ) ) ;
#58503=CARTESIAN_POINT ( 'NONE',  ( 38.55722148433031293, -287.2222308513680673, -257.3084199529279203 ) ) ;
#58504=CARTESIAN_POINT ( 'NONE',  ( -64.91784471381103572, -279.3938877601074182, -339.7802786118872405 ) ) ;
#58506=CARTESIAN_POINT ( 'NONE',  ( -54.83618902055553690, -284.6172688549650616, -199.0268900767604521 ) ) ;
#58507=CARTESIAN_POINT ( 'NONE',  ( 8.606103754259725847, -284.6815505852092087, -211.0838039067718341 ) ) ;
#58508=CARTESIAN_POINT ( 'NONE',  ( -83.79068156146763613, -277.5621729979981751, -210.4382665843251630 ) ) ;
#58509=CARTESIAN_POINT ( 'NONE',  ( 180.5468918863934960, 256.3577768311903355, -167.2605672291198857 ) ) ;
#58510=CARTESIAN_POINT ( 'NONE',  ( -109.4808917354702942, -284.2133802210203726, -258.7092963028582631 ) ) ;
#58511=CARTESIAN_POINT ( 'NONE',  ( 10.56267706767602554, -281.9018561384991131, -210.5170636391363814 ) ) ;
#58512=CARTESIAN_POINT ( 'NONE',  ( 14.43613390439028699, -287.4040499083869236, -327.1065561166008138 ) ) ;
#58513=CARTESIAN_POINT ( 'NONE',  ( -53.93696164439098339, -278.8617389779533937, -344.7861343549371895 ) ) ;
#58514=CARTESIAN_POINT ( 'NONE',  ( -73.84670828488057737, -278.8416451607796489, -337.6120443397962276 ) ) ;
#58515=CARTESIAN_POINT ( 'NONE',  ( -107.2265035552686641, -278.6647991774414095, -249.2633869563441067 ) ) ;
#58516=CARTESIAN_POINT ( 'NONE',  ( -38.12434443258450045, -276.0221872799673406, -195.7204167890363351 ) ) ;
#58517=CARTESIAN_POINT ( 'NONE',  ( 20.37869045009978919, -292.8618381384318923, -219.3769307577513530 ) ) ;
#58518=CARTESIAN_POINT ( 'NONE',  ( 23.28316454167746485, -286.1676621772494400, -313.9096264323952141 ) ) ;
#58520=CARTESIAN_POINT ( 'NONE',  ( -25.16951929372627461, -293.8050023533035642, -195.1395889667691392 ) ) ;
#58521=CARTESIAN_POINT ( 'NONE',  ( 32.63779622284481263, -292.7607085117251700, -292.2036490686687671 ) ) ;
#58522=CARTESIAN_POINT ( 'NONE',  ( 6.072104311234774343, -294.1116789976222776, -329.1380894829464978 ) ) ;
#58524=CARTESIAN_POINT ( 'NONE',  ( -102.9585227589905685, -292.1531723257456861, -230.5607770174415805 ) ) ;
#58525=CARTESIAN_POINT ( 'NONE',  ( 24.22075796338032916, -282.7492417371565807, -309.8744442351149928 ) ) ;
#58526=CARTESIAN_POINT ( 'NONE',  ( -26.25142631353630662, -297.1082790415194950, -193.6722057268607671 ) ) ;
#58527=CARTESIAN_POINT ( 'NONE',  ( -107.6348193458637326, -290.8036565344600035, -301.6720160924972447 ) ) ;
#58528=CARTESIAN_POINT ( 'NONE',  ( -52.69091141803813372, -281.3862282238339958, -344.6084534189697592 ) ) ;
#58530=CARTESIAN_POINT ( 'NONE',  ( -60.01699755011050996, -289.6714918272361388, -343.9245272175650712 ) ) ;
#58531=CARTESIAN_POINT ( 'NONE',  ( -52.09735192134409232, -286.1912986017371736, -198.8463766571815370 ) ) ;
#58532=CARTESIAN_POINT ( 'NONE',  ( 5.216678999461890953, -58.13084686227820441, -354.5881712518272479 ) ) ;
#58533=CARTESIAN_POINT ( 'NONE',  ( 166.1111599400100545, 232.1286469159066712, -191.2976056663461861 ) ) ;
#58534=CARTESIAN_POINT ( 'NONE',  ( -97.95619041649757719, -246.4268646875643469, -331.2869283950922750 ) ) ;
#58535=CARTESIAN_POINT ( 'NONE',  ( -110.1256530495713690, -277.8534005582075679, -262.4534283055543824 ) ) ;
#58536=CARTESIAN_POINT ( 'NONE',  ( 9.484504338464780915, -279.6337342798196346, -213.8898574510124888 ) ) ;
#58537=CARTESIAN_POINT ( 'NONE',  ( -29.83672130469200567, -273.8114249045856923, -193.7489806650517039 ) ) ;
#58538=CARTESIAN_POINT ( 'NONE',  ( 123.0799137420843294, 147.2756895088847671, -261.2470527563303904 ) ) ;
#58539=CARTESIAN_POINT ( 'NONE',  ( -36.73883383678317216, -278.6343241528004455, -193.9397768056164466 ) ) ;
#58540=CARTESIAN_POINT ( 'NONE',  ( -29.29178007417424467, -280.9699065246471719, -344.6222300214747634 ) ) ;
#58541=CARTESIAN_POINT ( 'NONE',  ( -66.51440299236104181, -297.1891122513745245, -340.5387068283817484 ) ) ;
#58542=CARTESIAN_POINT ( 'NONE',  ( -52.38856171358685287, -292.3467078529504874, -198.8138550837406626 ) ) ;
#58543=CARTESIAN_POINT ( 'NONE',  ( -92.79477947521067449, -288.5532671139583272, -318.6678811918050656 ) ) ;
#58544=CARTESIAN_POINT ( 'NONE',  ( -30.49768110483991279, -298.6280333152058120, -193.4221014502348339 ) ) ;
#58545=CARTESIAN_POINT ( 'NONE',  ( -104.7630216196258743, -297.0941618583510149, -242.3724521904902360 ) ) ;
#58548=CARTESIAN_POINT ( 'NONE',  ( -112.9436993789136778, -280.4563983155761093, -271.6094741629862597 ) ) ;
#58550=CARTESIAN_POINT ( 'NONE',  ( 11.50158399539638232, -281.8285767952877450, -215.6933974442714543 ) ) ;
#58551=CARTESIAN_POINT ( 'NONE',  ( -107.7094822790085686, -279.9432180013292850, -299.0377504007761900 ) ) ;
#58552=CARTESIAN_POINT ( 'NONE',  ( -13.46394022879381858, -281.7932397158982099, -339.6482727907780941 ) ) ;
#58553=CARTESIAN_POINT ( 'NONE',  ( -27.17555842637023389, -272.6634384562116793, -197.3209871789000545 ) ) ;
#58556=CARTESIAN_POINT ( 'NONE',  ( 23.49870851570914354, -275.7270670020534453, -223.4078021316897491 ) ) ;
#58557=MANIFOLD_SOLID_BREP ( 'Shell2', #73378 ) ;
#58560=CARTESIAN_POINT ( 'NONE',  ( 37.62553841112938358, -277.5980497989574474, -273.9229055294348996 ) ) ;
#58561=CARTESIAN_POINT ( 'NONE',  ( -97.47651404494067151, -276.4918510350735232, -317.5035664825592221 ) ) ;
#58562=ORIENTED_EDGE ( 'NONE', *, *, #76364, .F. ) ;
#58564=CARTESIAN_POINT ( 'NONE',  ( 6.000033185988877804, -284.4478194515640439, -332.0682771191629286 ) ) ;
#58565=CARTESIAN_POINT ( 'NONE',  ( -96.88684040607151360, -290.3429516492303151, -227.7668782799815688 ) ) ;
#58567=CARTESIAN_POINT ( 'NONE',  ( -36.55812781050649107, -285.4103347906405475, -193.4540209268634783 ) ) ;
#58568=CARTESIAN_POINT ( 'NONE',  ( -23.90319559126147553, -281.1179765025152619, -343.1442245866483631 ) ) ;
#58569=CARTESIAN_POINT ( 'NONE',  ( -2.162823903857724162, -281.1515848506590487, -335.0115912743746662 ) ) ;
#58570=CARTESIAN_POINT ( 'NONE',  ( 12.10855575273215656, -284.8256454208595869, -214.6502524807501402 ) ) ;
#58571=CARTESIAN_POINT ( 'NONE',  ( 32.34880888967980894, -282.4512628904454914, -247.1714141487681502 ) ) ;
#58572=CARTESIAN_POINT ( 'NONE',  ( -77.74220388725862563, -271.5094251216670500, -207.1725118625857931 ) ) ;
#58573=CARTESIAN_POINT ( 'NONE',  ( -112.8100083746973468, -282.8141768368542444, -281.2689785234019269 ) ) ;
#58574=CARTESIAN_POINT ( 'NONE',  ( -37.65439156176088886, -297.0561888963941328, -345.3732096272007652 ) ) ;
#58575=CARTESIAN_POINT ( 'NONE',  ( -98.19578601263224016, -280.0585732387698386, -229.5256365944144363 ) ) ;
#58576=CARTESIAN_POINT ( 'NONE',  ( -86.56897677220887033, -287.3706700716140858, -213.4881093479861249 ) ) ;
#58579=CARTESIAN_POINT ( 'NONE',  ( 19.28303206256286728, -294.7816820182009678, -220.3120476382606228 ) ) ;
#58580=CARTESIAN_POINT ( 'NONE',  ( -95.16380222357950913, -275.8927509602522150, -318.1473996638956123 ) ) ;
#58581=CARTESIAN_POINT ( 'NONE',  ( 7.831303977691545626, -287.6500501471978168, -332.5842551510345970 ) ) ;
#58582=CARTESIAN_POINT ( 'NONE',  ( 36.22024433781560049, -292.0293028138454474, -276.2840176252884703 ) ) ;
#58583=CARTESIAN_POINT ( 'NONE',  ( -69.48210493171671942, -276.1690247434627281, -336.4676957458291895 ) ) ;
#58584=CARTESIAN_POINT ( 'NONE',  ( -95.40283238755658601, -295.3341532651323291, -224.1034655898878611 ) ) ;
#58585=CARTESIAN_POINT ( 'NONE',  ( -34.85727438330356875, -293.3991895667081735, -196.9099702185754097 ) ) ;
#58586=CARTESIAN_POINT ( 'NONE',  ( 31.95455697924148097, -283.6233781216988064, -236.9535640164627353 ) ) ;
#58588=CARTESIAN_POINT ( 'NONE',  ( -58.67620262530888908, -293.8029137561102857, -343.6797370096682585 ) ) ;
#58589=CARTESIAN_POINT ( 'NONE',  ( 33.43143252167217128, -288.8779464051774539, -249.3975920073466170 ) ) ;
#58590=CARTESIAN_POINT ( 'NONE',  ( -111.2819287127388037, -288.5693267298611318, -287.9330410642306219 ) ) ;
#58591=CARTESIAN_POINT ( 'NONE',  ( 24.74513969528323543, -289.5192455207957778, -309.8655384630407639 ) ) ;
#58593=CARTESIAN_POINT ( 'NONE',  ( -34.56164648202492629, -289.8193032128233426, -343.5194473649704605 ) ) ;
#58595=CARTESIAN_POINT ( 'NONE',  ( 12.17092328126948964, -289.5858704919950810, -328.8120276471631200 ) ) ;
#58596=CARTESIAN_POINT ( 'NONE',  ( -39.51402739835575062, -278.0451456051525838, -195.0244597577606100 ) ) ;
#58597=CARTESIAN_POINT ( 'NONE',  ( -77.48511365191963307, -279.8627412386069295, -204.6164518453301469 ) ) ;
#58598=CARTESIAN_POINT ( 'NONE',  ( 39.59853839682320853, -281.2493709843002989, -272.7991473443757400 ) ) ;
#58599=CARTESIAN_POINT ( 'NONE',  ( 37.65485837510035338, -285.5612182998773960, -271.0800465722693389 ) ) ;
#58600=CARTESIAN_POINT ( 'NONE',  ( -110.6019403019620171, -273.5598536869071609, -270.3739484367653745 ) ) ;
#58601=CARTESIAN_POINT ( 'NONE',  ( -94.01815770130332339, -277.3619936420787440, -222.3973899133826251 ) ) ;
#58602=CARTESIAN_POINT ( 'NONE',  ( -49.78737457124737631, -281.2106031406761417, -344.3737597120046985 ) ) ;
#58604=CARTESIAN_POINT ( 'NONE',  ( -84.45365961702597701, -276.1668855571060135, -330.4546906633462982 ) ) ;
#58605=CARTESIAN_POINT ( 'NONE',  ( -96.04262244044051045, -282.8050836573171409, -319.7341946126602465 ) ) ;
#58606=CARTESIAN_POINT ( 'NONE',  ( -108.0988892504093286, -273.6023889806285752, -251.5650875456485380 ) ) ;
#58607=CARTESIAN_POINT ( 'NONE',  ( -113.7531456745012690, -274.0130566916598696, -267.5337022576003960 ) ) ;
#58608=CARTESIAN_POINT ( 'NONE',  ( 16.54389171315690632, -275.9257658279097996, -319.6588741575004065 ) ) ;
#58609=CARTESIAN_POINT ( 'NONE',  ( 9.496526050936175523, -296.4087377645370793, -329.0041672289834196 ) ) ;
#58610=CARTESIAN_POINT ( 'NONE',  ( -89.48992366539307852, -289.9298306164640735, -327.0141213132939697 ) ) ;
#58611=CARTESIAN_POINT ( 'NONE',  ( 14.19733570862872618, -278.8487698430856767, -215.0352322596864951 ) ) ;
#58612=CARTESIAN_POINT ( 'NONE',  ( -70.89579604493113152, -291.4549373071619698, -201.0565535460021351 ) ) ;
#58613=CARTESIAN_POINT ( 'NONE',  ( -42.69303489604784829, -288.1799223578173610, -343.4514063856719304 ) ) ;
#58614=CARTESIAN_POINT ( 'NONE',  ( 5.451403755680182428, -292.4731416865045617, -332.0178163447873771 ) ) ;
#58617=CARTESIAN_POINT ( 'NONE',  ( -98.16537690546653039, -289.4981136238827162, -310.8619005052901230 ) ) ;
#58619=CARTESIAN_POINT ( 'NONE',  ( -63.13369544164111602, -286.6655033851706094, -198.0590212603191276 ) ) ;
#58620=CARTESIAN_POINT ( 'NONE',  ( -67.74223827176244583, -288.1233781216987495, -207.3071070584150277 ) ) ;
#58621=CARTESIAN_POINT ( 'NONE',  ( 22.97931751020588464, -293.2480101418277627, -317.8605678744572742 ) ) ;
#58622=CARTESIAN_POINT ( 'NONE',  ( 25.53465373807715721, -283.4470714877490423, -313.9715765906631759 ) ) ;
#58623=CARTESIAN_POINT ( 'NONE',  ( -59.97661420160818579, -285.5838041910504330, -200.9589518104834553 ) ) ;
#58624=CARTESIAN_POINT ( 'NONE',  ( 25.69022420480298408, -276.3497976632214659, -232.4707842078587419 ) ) ;
#58625=CARTESIAN_POINT ( 'NONE',  ( -38.39012820922796720, -293.0854690731818550, -344.9985590232853951 ) ) ;
#58626=CARTESIAN_POINT ( 'NONE',  ( -40.53833682900900470, -275.8881287627837082, -343.7010801597880914 ) ) ;
#58629=CARTESIAN_POINT ( 'NONE',  ( -16.51668032641892481, -294.4570496281735927, -344.5247878499865237 ) ) ;
#58630=CARTESIAN_POINT ( 'NONE',  ( -5.198574295426515945, -288.3985923036784129, -203.2044271127489026 ) ) ;
#58631=CARTESIAN_POINT ( 'NONE',  ( -112.3001062314025091, -297.4282858397923519, -286.5700619827166520 ) ) ;
#58632=CARTESIAN_POINT ( 'NONE',  ( -10.72057016878578040, -287.0601374721277352, -202.2652112457444673 ) ) ;
#58633=CARTESIAN_POINT ( 'NONE',  ( -56.87576311536285090, -276.3567077033968644, -344.6537351831965452 ) ) ;
#58634=CARTESIAN_POINT ( 'NONE',  ( -50.44198420407452232, -295.8664875174620761, -346.1889661637607674 ) ) ;
#58635=CARTESIAN_POINT ( 'NONE',  ( 9.446252132475636998, -286.5567105174837934, -330.0197317783017752 ) ) ;
#58636=CARTESIAN_POINT ( 'NONE',  ( 38.79625857030477221, -294.0273815859306978, -281.7081676768841021 ) ) ;
#58638=PLANE ( 'NONE',  #32667 ) ;
#58639=CARTESIAN_POINT ( 'NONE',  ( 193.6786666067652618, 275.6390347797879485, -124.0807961620095767 ) ) ;
#58640=CARTESIAN_POINT ( 'NONE',  ( -5.084794639619390821, -287.9892316847883649, -201.2076668493518810 ) ) ;
#58641=CARTESIAN_POINT ( 'NONE',  ( -88.47809603358389552, -288.9094976428775681, -206.1857440867352693 ) ) ;
#58643=CARTESIAN_POINT ( 'NONE',  ( -94.88000257100489421, -278.5928676406996942, -219.3448799917398446 ) ) ;
#58644=CARTESIAN_POINT ( 'NONE',  ( 35.10463050943396013, -283.7943648817204121, -289.1620979309058157 ) ) ;
#58645=CARTESIAN_POINT ( 'NONE',  ( 204.9738562186072670, 293.9637359089629172, -68.56503966176641995 ) ) ;
#58646=CARTESIAN_POINT ( 'NONE',  ( -108.4732631611209825, -283.4850257510628921, -242.3084064562328592 ) ) ;
#58647=CARTESIAN_POINT ( 'NONE',  ( 21.48058208509784350, -286.2623387316310755, -316.0025022166556141 ) ) ;
#58648=CARTESIAN_POINT ( 'NONE',  ( -38.36488130185693990, -275.8998640020965922, -194.6032234466659361 ) ) ;
#58650=CARTESIAN_POINT ( 'NONE',  ( -108.8406547349348585, -297.2433762930133412, -255.2713699362329010 ) ) ;
#58651=CARTESIAN_POINT ( 'NONE',  ( -0.5253180154882282071, -293.2370720750670898, -334.0257783518213728 ) ) ;
#58652=CARTESIAN_POINT ( 'NONE',  ( -88.86929690035373142, -280.0018916324025895, -213.2803019653650267 ) ) ;
#58653=CARTESIAN_POINT ( 'NONE',  ( -43.20708927548842837, -277.1282792697838886, -343.1251009009618542 ) ) ;
#58654=CARTESIAN_POINT ( 'NONE',  ( -107.7141891568926297, -278.1625026371798413, -250.5257187786494342 ) ) ;
#58655=CARTESIAN_POINT ( 'NONE',  ( -34.12995575822717598, -275.1713252126160114, -193.7375105987864856 ) ) ;
#58656=CARTESIAN_POINT ( 'NONE',  ( 12.49328479277501458, -275.2967510603361916, -328.6531996647869960 ) ) ;
#58658=CARTESIAN_POINT ( 'NONE',  ( 36.97544691305154174, -273.6863813148131044, -280.8278042308323279 ) ) ;
#58659=CARTESIAN_POINT ( 'NONE',  ( -102.6028375552395744, -297.4544252039078742, -310.1051770813055555 ) ) ;
#58660=DIRECTION ( 'NONE',  ( 0.000000000000000000, 0.000000000000000000, -1.000000000000000000 ) ) ;
#58661=CARTESIAN_POINT ( 'NONE',  ( -109.0101294763935016, -268.7602059993127455, -295.2240039188629339 ) ) ;
#58662=CARTESIAN_POINT ( 'NONE',  ( -22.41025438098025546, -287.3273920472772147, -198.5366155816941216 ) ) ;
#58663=CARTESIAN_POINT ( 'NONE',  ( -110.8884383366877415, -286.0694397909495592, -289.5137248042375973 ) ) ;
#58664=CARTESIAN_POINT ( 'NONE',  ( -46.72975171978337272, -285.2785392073601543, -197.8136710112836738 ) ) ;
#58665=CARTESIAN_POINT ( 'NONE',  ( -101.4973222647122668, -277.4461919903855005, -233.8851455921334548 ) ) ;
#58666=CARTESIAN_POINT ( 'NONE',  ( -79.05140265793581023, -285.4817698924738352, -331.7709396172847960 ) ) ;
#58667=CARTESIAN_POINT ( 'NONE',  ( -46.52383406957923739, -278.4135240327029805, -197.1904769732057048 ) ) ;
#58668=CARTESIAN_POINT ( 'NONE',  ( -7.368742320941616519, -277.7292432341420749, -337.2628957969927228 ) ) ;
#58670=CARTESIAN_POINT ( 'NONE',  ( 35.76051435095966724, -276.0605647392807214, -271.5797414414307696 ) ) ;
#58671=CARTESIAN_POINT ( 'NONE',  ( 1.283936995486041344, -281.3567960196212994, -203.8760080598230218 ) ) ;
#58672=CARTESIAN_POINT ( 'NONE',  ( 28.25581962852276519, -282.5713643484444901, -310.6677197834216599 ) ) ;
#58676=CARTESIAN_POINT ( 'NONE',  ( -51.43198739208584414, -291.0909083632765260, -344.8041786581816837 ) ) ;
#58677=CARTESIAN_POINT ( 'NONE',  ( -98.64410457595269577, -288.6238502468863771, -316.1573824283742624 ) ) ;
#58678=CARTESIAN_POINT ( 'NONE',  ( -105.9537099180454618, -296.0889554714380552, -244.8183167242063121 ) ) ;
#58680=CARTESIAN_POINT ( 'NONE',  ( -70.84579838389640827, -290.9702826215589084, -201.1455981385965686 ) ) ;
#58681=CARTESIAN_POINT ( 'NONE',  ( 14.55807695652621270, -286.7851824383562303, -322.6786187862156225 ) ) ;
#58683=CARTESIAN_POINT ( 'NONE',  ( 35.35578512918814909, -288.8910776122786501, -280.5624664279043827 ) ) ;
#58684=CARTESIAN_POINT ( 'NONE',  ( -106.6379572354042296, -292.6233781216987495, -303.7686719486574702 ) ) ;
#58685=CARTESIAN_POINT ( 'NONE',  ( 31.05176525278180577, -289.9559266763461096, -301.1399181365704862 ) ) ;
#58686=CARTESIAN_POINT ( 'NONE',  ( -41.68080614407671902, -287.1065093820386664, -345.4153511425020611 ) ) ;
#58687=CARTESIAN_POINT ( 'NONE',  ( -107.9849569948173382, -285.2385268511987420, -289.7200563243366105 ) ) ;
#58688=CARTESIAN_POINT ( 'NONE',  ( -106.0450824460865675, -292.1521867671137329, -300.9828664745254514 ) ) ;
#58689=CARTESIAN_POINT ( 'NONE',  ( 82.16214272339226454, -298.5110651170496112, -193.6458011586250620 ) ) ;
#58691=CARTESIAN_POINT ( 'NONE',  ( -33.45209830827303676, -300.0206301958165795, -194.7998491850339349 ) ) ;
#58692=CARTESIAN_POINT ( 'NONE',  ( 14.03080343361200910, -281.5058699449105006, -322.5233926421246906 ) ) ;
#58693=CARTESIAN_POINT ( 'NONE',  ( -104.8230045105705557, -282.1193390145845115, -303.2107995657173660 ) ) ;
#58694=CARTESIAN_POINT ( 'NONE',  ( 34.29724498811630440, -293.1020786641420841, -298.1463723948273810 ) ) ;
#58695=CARTESIAN_POINT ( 'NONE',  ( -107.2563597055038969, -271.1106076826631011, -246.0729647200678869 ) ) ;
#58696=CARTESIAN_POINT ( 'NONE',  ( 35.57016313946201080, -273.8261203508047288, -285.3669300508146875 ) ) ;
#58697=CARTESIAN_POINT ( 'NONE',  ( -110.2918884991095609, -297.7451608369148062, -279.6849122192661525 ) ) ;
#58699=CARTESIAN_POINT ( 'NONE',  ( -36.92458206176511482, -272.6320452602067235, -193.9385305194504951 ) ) ;
#58700=CARTESIAN_POINT ( 'NONE',  ( -107.9387177782732010, -295.1549413519128393, -242.1122626865557095 ) ) ;
#58701=CARTESIAN_POINT ( 'NONE',  ( -20.69739856007482004, -296.2596851056119931, -342.0958768259982321 ) ) ;
#58703=CARTESIAN_POINT ( 'NONE',  ( -41.03717211239619900, -295.9026467098473177, -343.4417992770300998 ) ) ;
#58704=CARTESIAN_POINT ( 'NONE',  ( -112.3417001280820386, -272.5521521680024648, -270.3611179825637691 ) ) ;
#58705=CARTESIAN_POINT ( 'NONE',  ( -112.7106217909955319, -282.5414612805869865, -272.7709295338436277 ) ) ;
#58706=CARTESIAN_POINT ( 'NONE',  ( -95.28906866339589499, -297.1769671618695838, -225.9436502477421129 ) ) ;
#58707=CARTESIAN_POINT ( 'NONE',  ( -112.9982418408954885, -284.7346790332960040, -255.7628116991040201 ) ) ;
#58708=CARTESIAN_POINT ( 'NONE',  ( -24.74903386559984497, -284.8129953649403774, -344.9175061051861348 ) ) ;
#58710=CARTESIAN_POINT ( 'NONE',  ( 39.32600644743844498, -287.3053680525313780, -277.2753829408665069 ) ) ;
#58711=CARTESIAN_POINT ( 'NONE',  ( -32.00166042297281166, -290.1194948919369949, -195.7056164148254709 ) ) ;
#58712=CARTESIAN_POINT ( 'NONE',  ( -112.8356090845500574, -277.9295698575354550, -255.9789674237104009 ) ) ;
#58713=CARTESIAN_POINT ( 'NONE',  ( -4.829096099716524648, -280.1237833571632336, -337.9475929042657754 ) ) ;
#58715=CARTESIAN_POINT ( 'NONE',  ( -5.613176773358834915, -285.2738687217776601, -204.1624310261117330 ) ) ;
#58716=CARTESIAN_POINT ( 'NONE',  ( -111.6260730152491192, -289.2323913693102782, -289.4747624125574816 ) ) ;
#58717=DIRECTION ( 'NONE',  ( 1.000000000000000000, 0.000000000000000000, 0.000000000000000000 ) ) ;
#58718=CARTESIAN_POINT ( 'NONE',  ( -110.8490849169315169, -298.2451752035632921, -263.2425357576393026 ) ) ;
#58719=CARTESIAN_POINT ( 'NONE',  ( -112.6587840659604183, -280.1397681681479526, -257.4792252402149870 ) ) ;
#58720=CARTESIAN_POINT ( 'NONE',  ( -33.54350951435366568, -293.0247046419877393, -345.6333789947981359 ) ) ;
#58721=CARTESIAN_POINT ( 'NONE',  ( 32.25017604882551581, -281.5139557742043053, -292.6404277766109203 ) ) ;
#58722=CARTESIAN_POINT ( 'NONE',  ( -41.94343917727029947, -295.2751768993224459, -347.2758820249123346 ) ) ;
#58723=CARTESIAN_POINT ( 'NONE',  ( 8.948227545833848495, -284.7615441348500553, -210.6404616641188170 ) ) ;
#58724=CARTESIAN_POINT ( 'NONE',  ( -71.61615328812959547, -281.5995509780946691, -203.6365573256980781 ) ) ;
#58725=CARTESIAN_POINT ( 'NONE',  ( -41.06312668853401959, -294.1588438930530174, -343.5144081940376850 ) ) ;
#58728=CARTESIAN_POINT ( 'NONE',  ( 33.53049388703569633, -283.2259544132777478, -246.7680799888565844 ) ) ;
#58729=CARTESIAN_POINT ( 'NONE',  ( -110.2733433894352686, -296.1171999221894566, -266.0063673927788841 ) ) ;
#58731=CARTESIAN_POINT ( 'NONE',  ( -85.28047601435909542, -276.9094976428776249, -210.1954327657594206 ) ) ;
#58732=CARTESIAN_POINT ( 'NONE',  ( -46.85086058707742040, -273.1314872313794240, -194.1132676026062427 ) ) ;
#58735=CARTESIAN_POINT ( 'NONE',  ( -94.28957238991719692, -291.0311551039254709, -224.6691645873775940 ) ) ;
#58736=CARTESIAN_POINT ( 'NONE',  ( -95.34849404617020241, -280.7072726407316168, -224.8884114915677515 ) ) ;
#58737=CARTESIAN_POINT ( 'NONE',  ( -0.1606389987241754747, -276.1556905325818434, -206.5967880756469128 ) ) ;
#58738=CARTESIAN_POINT ( 'NONE',  ( 11.00096335931202063, -283.9964246375881203, -329.3312574431718645 ) ) ;
#58739=CARTESIAN_POINT ( 'NONE',  ( -2.252258150526716296, -281.3717458410600329, -334.8414557679255950 ) ) ;
#58740=CARTESIAN_POINT ( 'NONE',  ( -39.18198955426010599, -279.0754116970554151, -345.3385411640683174 ) ) ;
#58742=CARTESIAN_POINT ( 'NONE',  ( -24.15751981521545488, -274.0492385822398660, -194.4440659278375563 ) ) ;
#58743=CARTESIAN_POINT ( 'NONE',  ( 2.358090243491804294, -296.4363192216363814, -333.3923367251136369 ) ) ;
#58746=CARTESIAN_POINT ( 'NONE',  ( 36.57356121965458584, -291.9039657184482621, -287.0580946508957254 ) ) ;
#58747=AXIS2_PLACEMENT_3D ( 'NONE', #52382, #67074, #59980 ) ;
#58748=CARTESIAN_POINT ( 'NONE',  ( -69.51241316975526274, -273.1245046829878902, -204.7636053447631923 ) ) ;
#58750=CARTESIAN_POINT ( 'NONE',  ( -22.34913209683123725, -293.7607615265937397, -195.4879632618886092 ) ) ;
#58751=CARTESIAN_POINT ( 'NONE',  ( -69.85430415644619018, -279.9805209788416391, -337.9475929042657754 ) ) ;
#58752=CARTESIAN_POINT ( 'NONE',  ( -73.26117819295754430, -292.7917612346524265, -202.6868537666159682 ) ) ;
#58753=CARTESIAN_POINT ( 'NONE',  ( -0.05642167294575807512, -290.5553912146856987, -335.3040271737373246 ) ) ;
#58754=CARTESIAN_POINT ( 'NONE',  ( 37.20693045233825558, -273.4607588499176813, -263.2717800785143822 ) ) ;
#58755=CARTESIAN_POINT ( 'NONE',  ( -77.10474928617466617, -279.5092683629496833, -333.3519622508209181 ) ) ;
#58756=CARTESIAN_POINT ( 'NONE',  ( 35.73339942444705741, -291.8155604207780129, -284.5506925276579864 ) ) ;
#58757=CARTESIAN_POINT ( 'NONE',  ( -28.39476240270343510, -282.0247845828132540, -195.0736700449982379 ) ) ;
#58759=CARTESIAN_POINT ( 'NONE',  ( -53.69853189574080687, -282.9344640767532724, -341.5788105460835027 ) ) ;
#58760=CARTESIAN_POINT ( 'NONE',  ( -96.58744848056015542, -280.2887644847710362, -221.6433232711877110 ) ) ;
#58761=CARTESIAN_POINT ( 'NONE',  ( -10.85381177139242403, -281.5093827006601828, -342.2951447254273489 ) ) ;
#58762=CARTESIAN_POINT ( 'NONE',  ( -97.73634555628086673, -278.8579922585502686, -317.7457886862556506 ) ) ;
#58764=CARTESIAN_POINT ( 'NONE',  ( 27.07403079322463668, -277.6143581862805831, -311.3656259189516504 ) ) ;
#58765=CARTESIAN_POINT ( 'NONE',  ( -21.33282851196159058, -285.3376638359844719, -340.3538533559490702 ) ) ;
#58768=CARTESIAN_POINT ( 'NONE',  ( -50.32449358500621628, -299.8865635524892923, -196.4933461189164632 ) ) ;
#58769=CARTESIAN_POINT ( 'NONE',  ( -68.75199337118469600, -275.4871800172071516, -338.0895803231078389 ) ) ;
#58770=CARTESIAN_POINT ( 'NONE',  ( -111.2715053261624973, -292.0890388265043498, -287.9768470182414717 ) ) ;
#58771=CARTESIAN_POINT ( 'NONE',  ( -20.04000514735208327, -291.6288750002951247, -199.2838207606529863 ) ) ;
#58772=CARTESIAN_POINT ( 'NONE',  ( 19.57449628544570430, -287.7641381107038683, -322.1501660396597231 ) ) ;
#58774=CARTESIAN_POINT ( 'NONE',  ( 38.64224064724579222, -292.0191144916779535, -261.8100281653390766 ) ) ;
#58775=CARTESIAN_POINT ( 'NONE',  ( -83.30875802780741424, -282.0935637074011879, -328.1629184752833339 ) ) ;
#58776=CARTESIAN_POINT ( 'NONE',  ( -95.91071519575355353, -291.7803499911562426, -315.9945386638127047 ) ) ;
#58777=CARTESIAN_POINT ( 'NONE',  ( -97.91490516879137829, -283.6115695659032099, -228.3674661123548049 ) ) ;
#58778=CARTESIAN_POINT ( 'NONE',  ( 28.60090835284257338, -283.3054247765423383, -302.9237864254142210 ) ) ;
#58779=CARTESIAN_POINT ( 'NONE',  ( -87.22241725032165505, -290.6685511483703976, -328.7810283087312655 ) ) ;
#58780=CARTESIAN_POINT ( 'NONE',  ( 20.56085653619570763, -281.4177116615019827, -225.7842793140839888 ) ) ;
#58781=CARTESIAN_POINT ( 'NONE',  ( 13.02897779753327079, -291.5326502509920488, -212.6480040234442299 ) ) ;
#58782=CARTESIAN_POINT ( 'NONE',  ( -2.305675900842721227, -287.3066541688756956, -201.9604641642754359 ) ) ;
#58783=CARTESIAN_POINT ( 'NONE',  ( 35.78857806957747556, -287.7415676724920104, -246.2849360227185116 ) ) ;
#58784=CARTESIAN_POINT ( 'NONE',  ( -57.39642358597571103, -285.9528206369439545, -200.1172791368904313 ) ) ;
#58787=CARTESIAN_POINT ( 'NONE',  ( 8.183167501695949753, -296.2972575327050890, -330.9234157028564596 ) ) ;
#58788=CARTESIAN_POINT ( 'NONE',  ( -113.7424321250618249, -295.1749299433818692, -275.2907988800445196 ) ) ;
#58789=CARTESIAN_POINT ( 'NONE',  ( -105.4911208791931330, -277.2534491571777835, -297.1765034712289548 ) ) ;
#58790=CARTESIAN_POINT ( 'NONE',  ( -37.59898510129450955, -297.3976003181313672, -193.4634808821086267 ) ) ;
#58791=CARTESIAN_POINT ( 'NONE',  ( 19.89643698911766023, -291.3813244230000805, -223.9245243118323287 ) ) ;
#58792=CARTESIAN_POINT ( 'NONE',  ( -6.121646524917198740, -276.2283127508886196, -203.2546185259684250 ) ) ;
#58793=CARTESIAN_POINT ( 'NONE',  ( -106.9477354740237445, -294.4596834732561774, -295.6709159691966988 ) ) ;
#58794=CARTESIAN_POINT ( 'NONE',  ( 16.46059319169603441, -295.4708789818221817, -320.2854981851360776 ) ) ;
#58795=CARTESIAN_POINT ( 'NONE',  ( 1.746232537962481013, -295.5959720133897690, -332.4402717917050154 ) ) ;
#58797=CARTESIAN_POINT ( 'NONE',  ( -78.49503503040311614, -293.6046204367660835, -333.2612885011664048 ) ) ;
#58798=CARTESIAN_POINT ( 'NONE',  ( -107.1689386346646131, -298.9101366648176850, -242.8500217586268377 ) ) ;
#58799=CARTESIAN_POINT ( 'NONE',  ( -105.3270168392380697, -291.1285187111868140, -297.7259222133938579 ) ) ;
#58800=CARTESIAN_POINT ( 'NONE',  ( -88.51363961834874772, -296.1270039214653025, -322.5236324848327740 ) ) ;
#58801=CARTESIAN_POINT ( 'NONE',  ( -103.5188299238998297, -280.0554358438674285, -306.4026813794088184 ) ) ;
#58802=CARTESIAN_POINT ( 'NONE',  ( -94.58163516429823403, -277.9292140568590526, -219.5980594611044694 ) ) ;
#58804=CARTESIAN_POINT ( 'NONE',  ( -97.72786026384194713, -272.5383926024172183, -222.7499380851481021 ) ) ;
#58805=CARTESIAN_POINT ( 'NONE',  ( 1.838847016384126176, -280.6038627548596764, -333.7158386789578799 ) ) ;
#58806=CARTESIAN_POINT ( 'NONE',  ( -111.6173244878300466, -277.1670840823454114, -253.3443014483818274 ) ) ;
#58807=CARTESIAN_POINT ( 'NONE',  ( -40.89560963756561307, -278.0074011126604887, -195.2656276319985693 ) ) ;
#58808=CARTESIAN_POINT ( 'NONE',  ( -110.9309288753746898, -271.1271092316917475, -270.3430129928519818 ) ) ;
#58809=CARTESIAN_POINT ( 'NONE',  ( 26.16589086450915147, -277.0148976564033205, -230.3685084577820703 ) ) ;
#58812=CARTESIAN_POINT ( 'NONE',  ( -110.0392043883640554, -288.8266985274099170, -250.4758942532522781 ) ) ;
#58813=CARTESIAN_POINT ( 'NONE',  ( -69.35730438698212197, -289.4618734955298578, -340.4041149107267756 ) ) ;
#58814=CARTESIAN_POINT ( 'NONE',  ( 16.75210782339269855, -276.8195081143772427, -218.0955442132021744 ) ) ;
#58815=CARTESIAN_POINT ( 'NONE',  ( -35.74177478704485367, -296.0720672345574940, -195.5283229024749687 ) ) ;
#58816=CARTESIAN_POINT ( 'NONE',  ( -46.47613981931052507, -285.1361935216064012, -194.0674692839361342 ) ) ;
#58818=CARTESIAN_POINT ( 'NONE',  ( 33.32110402717074038, -279.8794175166545983, -295.6474551530456552 ) ) ;
#58820=CARTESIAN_POINT ( 'NONE',  ( 27.84619894006351259, -291.8908784391032896, -236.6317788436040246 ) ) ;
#58821=CARTESIAN_POINT ( 'NONE',  ( -70.51346805374795679, -283.7497013960384606, -203.9353496555264371 ) ) ;
#58824=CARTESIAN_POINT ( 'NONE',  ( 36.45556163586699228, -291.3793049181351762, -256.9118003839631683 ) ) ;
#58825=CARTESIAN_POINT ( 'NONE',  ( -43.25105288263891623, -278.7281494628791734, -343.9241519424434728 ) ) ;
#58826=CARTESIAN_POINT ( 'NONE',  ( -102.5718806867889157, -285.2295562291566284, -310.5236908862099767 ) ) ;
#58827=CARTESIAN_POINT ( 'NONE',  ( -16.15719934957107995, -272.4036582613009045, -197.7772889889810131 ) ) ;
#58828=CARTESIAN_POINT ( 'NONE',  ( -65.09322017174044106, -285.6793118563542180, -202.7880304802292244 ) ) ;
#58829=CARTESIAN_POINT ( 'NONE',  ( 30.71286712240053518, -276.6035724799260151, -242.2282736131600132 ) ) ;
#58830=CARTESIAN_POINT ( 'NONE',  ( -21.60835272250183792, -277.6482301879192391, -341.8629542140679973 ) ) ;
#58831=CARTESIAN_POINT ( 'NONE',  ( -103.9947421547751674, -286.0959762084872295, -304.8600033902848736 ) ) ;
#58834=CARTESIAN_POINT ( 'NONE',  ( -114.2339486883503525, -296.3232390150516267, -275.3372576180619831 ) ) ;
#58835=CARTESIAN_POINT ( 'NONE',  ( 14.25876389451109638, -288.7609432617553580, -216.3524702753543636 ) ) ;
#58837=CARTESIAN_POINT ( 'NONE',  ( -111.2869819898779866, -275.4805209788415823, -234.7871824221999191 ) ) ;
#58838=CARTESIAN_POINT ( 'NONE',  ( -105.8930810127271656, -277.9178965313490721, -235.8597397996663290 ) ) ;
#58840=CARTESIAN_POINT ( 'NONE',  ( -90.21600432072389708, -289.7196670843477477, -215.4176193140183670 ) ) ;
#58841=CARTESIAN_POINT ( 'NONE',  ( -27.76544216599693726, -287.6960984288273835, -197.2926361664710555 ) ) ;
#58843=CARTESIAN_POINT ( 'NONE',  ( -97.23878091489238784, -280.9124018662243429, -226.8833796760500832 ) ) ;
#58844=CARTESIAN_POINT ( 'NONE',  ( 14.21959363584990932, -289.7701931812119938, -326.8246708749955474 ) ) ;
#58845=CARTESIAN_POINT ( 'NONE',  ( -112.2268251196354498, -286.6165758677043414, -265.3564490736544599 ) ) ;
#58846=CARTESIAN_POINT ( 'NONE',  ( -67.70665367776241794, -277.6064314581030317, -341.1210614565739547 ) ) ;
#58847=CARTESIAN_POINT ( 'NONE',  ( -111.7048106414051176, -270.6597741438939124, -261.9851869764115122 ) ) ;
#58848=CARTESIAN_POINT ( 'NONE',  ( -114.2107287594964191, -278.4416154957397112, -265.8719708753156965 ) ) ;
#58849=CARTESIAN_POINT ( 'NONE',  ( -104.3297122676974737, -274.8380146674984985, -238.3693736255214048 ) ) ;
#58851=CARTESIAN_POINT ( 'NONE',  ( -114.2704648735229114, -293.0519495502703080, -270.3937649182068981 ) ) ;
#58852=CARTESIAN_POINT ( 'NONE',  ( -87.35236720989755099, -271.6062313604928136, -213.0818519771601132 ) ) ;
#58854=CARTESIAN_POINT ( 'NONE',  ( -107.2842172096729172, -278.3391845951010168, -249.2416306304934892 ) ) ;
#58855=CARTESIAN_POINT ( 'NONE',  ( -9.342588710788406914, -277.8992396139075822, -341.6637019363044487 ) ) ;
#58856=CARTESIAN_POINT ( 'NONE',  ( -33.08381711170639505, -282.0585357233502464, -347.0207434526104180 ) ) ;
#58857=CARTESIAN_POINT ( 'NONE',  ( 1.867139148768091284, -290.2798351753844486, -333.1356425550720246 ) ) ;
#58858=CARTESIAN_POINT ( 'NONE',  ( -82.57529162147292823, -298.9671753574708077, -208.8411628457500058 ) ) ;
#58859=CARTESIAN_POINT ( 'NONE',  ( -36.56115842718850928, -299.2667895415283397, -193.7580317958743024 ) ) ;
#58860=CARTESIAN_POINT ( 'NONE',  ( 25.99212602163962060, -296.0905427348685066, -310.3189504394732694 ) ) ;
#58861=CARTESIAN_POINT ( 'NONE',  ( 35.42707195648210217, -279.7773365963826677, -287.8721973614415219 ) ) ;
#58862=CARTESIAN_POINT ( 'NONE',  ( -38.07375235313784856, -272.0630438585761226, -195.7199034539361264 ) ) ;
#58863=CARTESIAN_POINT ( 'NONE',  ( 19.67446189663232659, -288.4595402276223695, -219.7303333684118343 ) ) ;
#58864=CARTESIAN_POINT ( 'NONE',  ( 6.016423568887450557, -287.3689832375177389, -329.5369704759186220 ) ) ;
#58865=CARTESIAN_POINT ( 'NONE',  ( 181.6150490960993409, 253.0111652753101907, -166.4923282781097384 ) ) ;
#58867=CARTESIAN_POINT ( 'NONE',  ( 26.93920550320910579, -286.6741355203776607, -311.7693127202081200 ) ) ;
#58868=CARTESIAN_POINT ( 'NONE',  ( -58.69936711498971249, -289.0026843312401184, -340.2418521902753810 ) ) ;
#58869=ORIENTED_EDGE ( 'NONE', *, *, #49629, .F. ) ;
#58870=CARTESIAN_POINT ( 'NONE',  ( -40.81628656781045805, -287.0892088255094450, -193.6969965600665375 ) ) ;
#58871=CARTESIAN_POINT ( 'NONE',  ( -41.85365194326441696, -277.4438183483711668, -343.2553328600326381 ) ) ;
#58872=CARTESIAN_POINT ( 'NONE',  ( 38.05083012601117076, -292.6498234575138895, -284.4840148903589920 ) ) ;
#58873=CARTESIAN_POINT ( 'NONE',  ( 0.8249828439521571521, -283.2083820463604411, -337.1342299560292304 ) ) ;
#58874=CARTESIAN_POINT ( 'NONE',  ( -6.528251926897602253, -281.9695935441709480, -200.5383867449178865 ) ) ;
#58875=CARTESIAN_POINT ( 'NONE',  ( -69.17383618124584643, -283.7928009957932431, -340.4644669373690817 ) ) ;
#58877=CARTESIAN_POINT ( 'NONE',  ( -38.35841236828841261, -280.3723462835667419, -197.3346479459443401 ) ) ;
#58878=CARTESIAN_POINT ( 'NONE',  ( -85.28047601435909542, -276.9094976428776249, -210.1954327657594206 ) ) ;
#58879=CARTESIAN_POINT ( 'NONE',  ( -77.88764424958249322, -208.6185847378275753, -357.2361643103192250 ) ) ;
#58880=CARTESIAN_POINT ( 'NONE',  ( -95.00277939147495943, -279.8924247011059379, -318.0805402447278425 ) ) ;
#58881=CARTESIAN_POINT ( 'NONE',  ( -96.26398026058502921, -239.2304635698770596, -341.1080143852184392 ) ) ;
#58882=CARTESIAN_POINT ( 'NONE',  ( 201.0615148111058659, 293.2992890834858599, -53.99999999998998845 ) ) ;
#58883=CARTESIAN_POINT ( 'NONE',  ( -51.58290462532085030, -273.0626169235216025, -198.5471792455737727 ) ) ;
#58884=CARTESIAN_POINT ( 'NONE',  ( 26.44539895100070481, -292.4914513847094781, -227.2472432484072158 ) ) ;
#58885=CARTESIAN_POINT ( 'NONE',  ( 65.71733346673669018, 45.99507470247991847, -315.6009874211030137 ) ) ;
#58886=CARTESIAN_POINT ( 'NONE',  ( -37.58741160275177151, -296.6238665303497442, -193.9507396201146889 ) ) ;
#58887=CARTESIAN_POINT ( 'NONE',  ( -7.918068316848774657, -287.0600984320034286, -338.0965385527741773 ) ) ;
#58888=CARTESIAN_POINT ( 'NONE',  ( -76.28622154589834281, -297.4387637551195667, -333.6206400863862314 ) ) ;
#58889=CARTESIAN_POINT ( 'NONE',  ( 33.13817507458800549, -288.5930380422211670, -249.4881567817710675 ) ) ;
#58891=CARTESIAN_POINT ( 'NONE',  ( -79.33818940139086351, -296.5455590026169261, -334.6193089097985194 ) ) ;
#58892=CARTESIAN_POINT ( 'NONE',  ( -27.83474727839874774, -286.6684892426094962, -197.9207543095453445 ) ) ;
#58893=CARTESIAN_POINT ( 'NONE',  ( 7.714195481699801960, -297.3993742180124400, -193.7671669734811530 ) ) ;
#58894=CARTESIAN_POINT ( 'NONE',  ( -40.63575174420508773, -292.8145727743919906, -193.5800792851728147 ) ) ;
#58895=CARTESIAN_POINT ( 'NONE',  ( 32.17710917916402735, -294.4686750548817145, -303.4498905156735873 ) ) ;
#58896=CARTESIAN_POINT ( 'NONE',  ( -72.62881040321610726, -291.7381120840700532, -206.3995418752397768 ) ) ;
#58898=CARTESIAN_POINT ( 'NONE',  ( -109.6660728353854211, -274.7541755011000078, -248.3074431420216115 ) ) ;
#58899=CARTESIAN_POINT ( 'NONE',  ( 38.33773321966071990, -274.1969360720172517, -258.4176196307475379 ) ) ;
#58901=CARTESIAN_POINT ( 'NONE',  ( -59.65315930053900217, -276.8412712734797765, -343.9934864945411732 ) ) ;
#58902=CARTESIAN_POINT ( 'NONE',  ( -108.7084954828143282, -271.1998180051596137, -251.3711846281036628 ) ) ;
#58903=CARTESIAN_POINT ( 'NONE',  ( -64.81189032102298597, -275.5541994271221142, -339.3813183339466946 ) ) ;
#58904=CARTESIAN_POINT ( 'NONE',  ( -46.22983261089778750, -275.0164206954806332, -197.5928063750375827 ) ) ;
#58905=CARTESIAN_POINT ( 'NONE',  ( -110.1209284606944152, -273.6007124993415687, -262.2007030896518245 ) ) ;
#58906=CARTESIAN_POINT ( 'NONE',  ( -107.1554795946085221, -274.7010474325054474, -240.2277889138057390 ) ) ;
#58907=CARTESIAN_POINT ( 'NONE',  ( -20.51837627309085477, -274.8573997149402999, -343.8679314951482979 ) ) ;
#58908=CARTESIAN_POINT ( 'NONE',  ( -75.70449723772257755, -296.2299559285264081, -332.6470406701505453 ) ) ;
#58909=CARTESIAN_POINT ( 'NONE',  ( 1.868557943611208305, -293.0914319994585071, -332.6944925141015119 ) ) ;
#58911=CARTESIAN_POINT ( 'NONE',  ( -77.77722091240910629, -278.0717534652443419, -335.8790847320632906 ) ) ;
#58912=CARTESIAN_POINT ( 'NONE',  ( -14.06745114323619994, -274.5293442224414662, -201.1707332554465495 ) ) ;
#58913=CARTESIAN_POINT ( 'NONE',  ( -60.34558280998903257, -284.4449287181309387, -197.3393371099973024 ) ) ;
#58914=CARTESIAN_POINT ( 'NONE',  ( -93.27002073957315531, -297.8540675986060933, -320.6003165645169020 ) ) ;
#58916=CARTESIAN_POINT ( 'NONE',  ( -17.11745018910179894, -285.5170379074419316, -199.9975442642219150 ) ) ;
#58917=CARTESIAN_POINT ( 'NONE',  ( -108.5877533675832609, -277.0539537357707331, -250.2649094742505724 ) ) ;
#58918=CARTESIAN_POINT ( 'NONE',  ( -110.4918092254458202, -277.0159210547054158, -278.8398254466879962 ) ) ;
#58919=CARTESIAN_POINT ( 'NONE',  ( -111.0342782519586535, -286.7322029505577916, -256.3507368174655880 ) ) ;
#58920=CARTESIAN_POINT ( 'NONE',  ( -16.54275820508942729, -275.5319100150848044, -199.9196723137866343 ) ) ;
#58922=CARTESIAN_POINT ( 'NONE',  ( 22.87321032881527927, -274.5823657021647932, -317.0792212899704623 ) ) ;
#58923=CARTESIAN_POINT ( 'NONE',  ( -97.96472585476233519, -281.1571022409814304, -225.8997953493799287 ) ) ;
#58925=CARTESIAN_POINT ( 'NONE',  ( 30.12485052753528691, -289.0261334428945474, -236.3379091713467801 ) ) ;
#58927=CARTESIAN_POINT ( 'NONE',  ( -0.2253787972388012761, -290.5452444218242931, -205.1311799287882423 ) ) ;
#58929=CARTESIAN_POINT ( 'NONE',  ( -99.69004999088407715, -271.7704218601475645, -231.4519063876864209 ) ) ;
#58930=CARTESIAN_POINT ( 'NONE',  ( -52.60091212836192653, -289.9943232883415476, -197.6583465907052641 ) ) ;
#58931=CARTESIAN_POINT ( 'NONE',  ( -87.71122462277782006, -229.8683413793775117, -344.1918058839762011 ) ) ;
#58932=CARTESIAN_POINT ( 'NONE',  ( -41.96691551842204859, -295.9936855049469386, -195.5038669475833615 ) ) ;
#58933=CARTESIAN_POINT ( 'NONE',  ( -5.929753362886146739, -287.1265573385318248, -339.9024535689309801 ) ) ;
#58934=CARTESIAN_POINT ( 'NONE',  ( -54.71092135828460812, -284.0717335456884598, -196.3862292355044303 ) ) ;
#58935=CARTESIAN_POINT ( 'NONE',  ( -96.38372556260050317, -285.3662044427798605, -314.2862150345133045 ) ) ;
#58936=CARTESIAN_POINT ( 'NONE',  ( 14.04536185640826140, -283.1112763957603988, -322.5090513385317763 ) ) ;
#58938=CARTESIAN_POINT ( 'NONE',  ( -77.24360547928358756, -291.5637579885327000, -334.3457171614279559 ) ) ;
#58940=CARTESIAN_POINT ( 'NONE',  ( -93.15975833594943367, -273.6102592397122635, -217.3316112663529793 ) ) ;
#58942=CARTESIAN_POINT ( 'NONE',  ( 22.13848541245901558, -286.2669767911008307, -316.9804598304331762 ) ) ;
#58943=CARTESIAN_POINT ( 'NONE',  ( 22.75835106102748284, -274.9071595080717429, -222.2051508334540415 ) ) ;
#58945=CARTESIAN_POINT ( 'NONE',  ( 22.66338385601455485, -296.1407979237416725, -314.7597294620327943 ) ) ;
#58947=CARTESIAN_POINT ( 'NONE',  ( -110.4683760289727132, -299.2662352645559167, -253.7030783399848985 ) ) ;
#58948=CARTESIAN_POINT ( 'NONE',  ( -16.00521877666289683, -281.4551766739191407, -340.6889079416566233 ) ) ;
#58949=CARTESIAN_POINT ( 'NONE',  ( -111.9498558912070649, -276.4295217776416962, -279.9204617637812476 ) ) ;
#58950=CARTESIAN_POINT ( 'NONE',  ( -41.13872418729586400, -272.4851975925565739, -194.0971875971027885 ) ) ;
#58951=CARTESIAN_POINT ( 'NONE',  ( 32.99366675342397315, -275.1642690305820906, -290.3274708819642456 ) ) ;
#58952=CARTESIAN_POINT ( 'NONE',  ( 11.37477944881166003, -294.2617961111847080, -214.9991687206116637 ) ) ;
#58953=CARTESIAN_POINT ( 'NONE',  ( 23.53017672154262740, -293.9297270521788619, -229.6422887141216336 ) ) ;
#58954=CARTESIAN_POINT ( 'NONE',  ( -110.4252592086296829, -286.4655049725199092, -258.5859294606688650 ) ) ;
#58955=CARTESIAN_POINT ( 'NONE',  ( 36.89193095903815589, -295.2063259400989637, -288.5259821930274029 ) ) ;
#58956=CARTESIAN_POINT ( 'NONE',  ( 37.59099979720906504, -295.0616616678769333, -285.8009611269818606 ) ) ;
#58957=CARTESIAN_POINT ( 'NONE',  ( -105.8050899075722242, -296.7250055449352431, -244.8822574279839728 ) ) ;
#58958=CARTESIAN_POINT ( 'NONE',  ( -93.90371999971841888, -291.8680659380046905, -319.6904826566554334 ) ) ;
#58959=CARTESIAN_POINT ( 'NONE',  ( -71.73683551964978733, -283.6608152228989752, -339.2521527108037844 ) ) ;
#58960=CARTESIAN_POINT ( 'NONE',  ( -67.57832461212092312, -295.7385586132759840, -201.0590153170460894 ) ) ;
#58961=CARTESIAN_POINT ( 'NONE',  ( -113.4871014224534207, -284.5329444566350503, -258.5694012711036862 ) ) ;
#58962=CARTESIAN_POINT ( 'NONE',  ( -36.42115123335905480, -279.0204850422260279, -345.0129935741259715 ) ) ;
#58963=EDGE_CURVE ( 'NONE', #42078, #14296, #48645, .T. ) ;
#58964=CARTESIAN_POINT ( 'NONE',  ( -95.26098864176314862, -283.9790968634272303, -225.2576083044342568 ) ) ;
#58965=CARTESIAN_POINT ( 'NONE',  ( 27.17011911388962631, -286.0636770660341313, -308.6132528892103437 ) ) ;
#58966=CARTESIAN_POINT ( 'NONE',  ( -20.01529863951607879, -278.4119629748929583, -196.5501794976063081 ) ) ;
#58967=CARTESIAN_POINT ( 'NONE',  ( 60.10016229265469434, 49.69813606028536412, -316.8989054076328671 ) ) ;
#58968=CARTESIAN_POINT ( 'NONE',  ( -109.6722641815814256, -284.1956824531847587, -260.0519984572719636 ) ) ;
#58969=CARTESIAN_POINT ( 'NONE',  ( 38.03760809406004029, -282.9295741673332714, -284.0710867462686338 ) ) ;
#58970=CARTESIAN_POINT ( 'NONE',  ( -51.65322569755518600, -288.2896914087506843, -345.7799514937378262 ) ) ;
#58971=CARTESIAN_POINT ( 'NONE',  ( 3.094430122261770499, -278.1192837331672081, -335.0093045963768077 ) ) ;
#58972=CARTESIAN_POINT ( 'NONE',  ( -28.64038288085472672, -278.2593049187998417, -346.4247803407751007 ) ) ;
#58973=CARTESIAN_POINT ( 'NONE',  ( -106.4440393492983361, -278.7000825332641512, -246.6715273318023662 ) ) ;
#58974=CARTESIAN_POINT ( 'NONE',  ( 25.71465333278364085, -294.1367638121599271, -314.5757150828541739 ) ) ;
#58975=CARTESIAN_POINT ( 'NONE',  ( 37.10069150266329530, -285.4536822671885830, -262.7218278711971493 ) ) ;
#58976=CARTESIAN_POINT ( 'NONE',  ( -33.59925002363613089, -293.6986446575913305, -194.2530731798775321 ) ) ;
#58977=CARTESIAN_POINT ( 'NONE',  ( -3.011119155476607467, -293.5075484080761612, -335.1348571395924409 ) ) ;
#58979=CARTESIAN_POINT ( 'NONE',  ( -4.330896837207037997, -294.2713237353578393, -335.5086316512798703 ) ) ;
#58980=CARTESIAN_POINT ( 'NONE',  ( -110.4828615250422672, -291.3388655520912494, -293.5966631804272993 ) ) ;
#58981=CARTESIAN_POINT ( 'NONE',  ( -4.308920300665096015, -281.1509040530035008, -205.1342636821833878 ) ) ;
#58982=CARTESIAN_POINT ( 'NONE',  ( -112.8346684315676214, -271.7890231973934760, -256.1623847164062227 ) ) ;
#58983=CARTESIAN_POINT ( 'NONE',  ( 38.99043517742371989, -288.3255484588295303, -280.1020315264777309 ) ) ;
#58984=CARTESIAN_POINT ( 'NONE',  ( 10.69093041217995577, -280.5364371622299018, -329.0222660641302923 ) ) ;
#58985=CARTESIAN_POINT ( 'NONE',  ( 16.67414502254573350, -288.6426288854995619, -325.2807812701290686 ) ) ;
#58986=CARTESIAN_POINT ( 'NONE',  ( -19.81488969910387610, -286.6170453603684791, -199.4746002033248260 ) ) ;
#58987=CARTESIAN_POINT ( 'NONE',  ( 189.2871950347832524, 271.4890288426949496, -139.5295763808702532 ) ) ;
#58988=CARTESIAN_POINT ( 'NONE',  ( -90.91305330213944558, -228.9931328718925272, -345.8290054490478269 ) ) ;
#58989=CARTESIAN_POINT ( 'NONE',  ( -93.95058081101505820, -238.6390622938258161, -338.4896325803341597 ) ) ;
#58990=CARTESIAN_POINT ( 'NONE',  ( -110.3302377797428164, -277.6740220409643598, -276.0813506845647112 ) ) ;
#58991=CARTESIAN_POINT ( 'NONE',  ( -110.4660108335609578, -277.5408090408507746, -265.1590744632180758 ) ) ;
#58992=CARTESIAN_POINT ( 'NONE',  ( -60.86062103588250949, -273.4219396883899549, -197.0074507838691602 ) ) ;
#58993=CARTESIAN_POINT ( 'NONE',  ( 203.9605228849236482, 292.2036489450777026, -53.99999999999079137 ) ) ;
#58994=CARTESIAN_POINT ( 'NONE',  ( -112.1370031990514207, -277.3246467595996023, -254.6689879938084289 ) ) ;
#58996=CARTESIAN_POINT ( 'NONE',  ( -67.79916128539190368, -297.2065701210532325, -339.9766124903949844 ) ) ;
#58997=CARTESIAN_POINT ( 'NONE',  ( -55.03332002274466106, -292.3107864874427264, -199.4739186658815981 ) ) ;
#58998=CARTESIAN_POINT ( 'NONE',  ( -44.03422780989043162, -274.9108829038041222, -193.8355570673414547 ) ) ;
#58999=CARTESIAN_POINT ( 'NONE',  ( -50.85848890386299104, -287.9131464509084708, -342.6526103191416723 ) ) ;
#59000=CARTESIAN_POINT ( 'NONE',  ( -87.97549789000325404, -274.0173976530444975, -212.4151804432509891 ) ) ;
#59001=CARTESIAN_POINT ( 'NONE',  ( -98.44873424958512942, -297.2733939395707807, -230.3330594901038353 ) ) ;
#59004=CARTESIAN_POINT ( 'NONE',  ( -58.91484553012831782, -281.6953376119867016, -197.9462466288546807 ) ) ;
#59006=CARTESIAN_POINT ( 'NONE',  ( -89.70395773035794207, -280.3720065990585226, -218.9820465119535982 ) ) ;
#59007=CARTESIAN_POINT ( 'NONE',  ( -101.0539782450407245, -280.8644320843680475, -228.8566927599659664 ) ) ;
#59008=CIRCLE ( 'NONE', #27241, 6.649382010133625620 ) ;
#59009=CARTESIAN_POINT ( 'NONE',  ( -66.06570792790306257, -272.1491368199127692, -202.4962586705537149 ) ) ;
#59012=CARTESIAN_POINT ( 'NONE',  ( 17.06139564414758780, -281.0224355033984693, -221.6856295421403900 ) ) ;
#59013=CARTESIAN_POINT ( 'NONE',  ( 3.424515937575832059, -277.3221164316823319, -335.5565000873030499 ) ) ;
#59014=CARTESIAN_POINT ( 'NONE',  ( 37.55540866634535035, -277.4904424956212665, -265.5422211869925491 ) ) ;
#59015=CARTESIAN_POINT ( 'NONE',  ( -64.89963812391857800, -275.9797482302329286, -341.6852499300943009 ) ) ;
#59018=CARTESIAN_POINT ( 'NONE',  ( 1.273400189806133120, -284.5189617964918511, -335.0703200330463574 ) ) ;
#59019=CARTESIAN_POINT ( 'NONE',  ( -66.61932730203763242, -290.8557044940275773, -203.3132076913531989 ) ) ;
#59020=CARTESIAN_POINT ( 'NONE',  ( -15.43454434066708991, -285.6769298719635231, -196.5942692700515977 ) ) ;
#59021=CARTESIAN_POINT ( 'NONE',  ( -111.4045987207254598, -282.7850627247556190, -270.8945385973955240 ) ) ;
#59022=CARTESIAN_POINT ( 'NONE',  ( -100.9192527532075303, -282.6223695539415530, -307.4187719590406687 ) ) ;
#59023=CARTESIAN_POINT ( 'NONE',  ( 34.42391937420377701, -285.3757675322946739, -250.5871437428761510 ) ) ;
#59024=CARTESIAN_POINT ( 'NONE',  ( -54.60096772788035935, -281.0306102546521743, -198.9696671825705607 ) ) ;
#59025=CARTESIAN_POINT ( 'NONE',  ( -94.48684376863917578, -271.2244966748070283, -221.7673554892992343 ) ) ;
#59026=CARTESIAN_POINT ( 'NONE',  ( -87.80713208062361730, -282.1430848468509680, -327.5252007734106883 ) ) ;
#59027=CARTESIAN_POINT ( 'NONE',  ( 26.41942082615214815, -296.0836441883024008, -309.9494991486461117 ) ) ;
#59028=CARTESIAN_POINT ( 'NONE',  ( -35.22598679939277844, -288.0787840986485548, -195.2113975730414666 ) ) ;
#59030=CARTESIAN_POINT ( 'NONE',  ( -50.34307550991074010, -293.8075671654117400, -195.9280713320153779 ) ) ;
#59031=CARTESIAN_POINT ( 'NONE',  ( 24.08975459295512067, -274.1370893516504452, -313.4755456552930468 ) ) ;
#59032=CARTESIAN_POINT ( 'NONE',  ( -82.76543319232921192, -288.8529912497588725, -332.3356554518549046 ) ) ;
#59033=CARTESIAN_POINT ( 'NONE',  ( 36.33472413660140887, -291.8857324229359165, -265.2813576249653806 ) ) ;
#59034=CARTESIAN_POINT ( 'NONE',  ( -97.29764994530189881, -276.6472350943205925, -312.8862461990938755 ) ) ;
#59035=CARTESIAN_POINT ( 'NONE',  ( -104.8318481053914439, -295.1032419795643591, -239.3191104695110027 ) ) ;
#59036=CARTESIAN_POINT ( 'NONE',  ( -84.99212525919708128, -291.0406806839543492, -326.3807604979632515 ) ) ;
#59039=CARTESIAN_POINT ( 'NONE',  ( -79.11374627568183371, -294.0845816161651669, -334.2188028154411086 ) ) ;
#59040=CARTESIAN_POINT ( 'NONE',  ( 24.92413337914894811, -289.6940734194641323, -309.9768521332014188 ) ) ;
#59041=CARTESIAN_POINT ( 'NONE',  ( -100.8248704200626662, -289.3494045767073999, -228.5071736212836129 ) ) ;
#59042=CARTESIAN_POINT ( 'NONE',  ( -58.84410339083934360, -290.7609546723720086, -340.7920499248559167 ) ) ;
#59044=CARTESIAN_POINT ( 'NONE',  ( -97.47581569208040264, -290.7754018532565965, -312.0543351086399184 ) ) ;
#59047=CARTESIAN_POINT ( 'NONE',  ( -48.79439720628084132, -290.3998488215689804, -346.1567423622017259 ) ) ;
#59048=CARTESIAN_POINT ( 'NONE',  ( -6.871820801296058434, -278.4701452238938373, -201.4269532034054748 ) ) ;
#59049=CARTESIAN_POINT ( 'NONE',  ( -48.12002027596228260, -280.2520172715671833, -194.0867388308380157 ) ) ;
#59050=CARTESIAN_POINT ( 'NONE',  ( -64.73083512763891179, -279.3709636644597936, -198.3634043056420069 ) ) ;
#59051=CARTESIAN_POINT ( 'NONE',  ( -70.85383957383592701, -283.6099794496257118, -203.2503172555763626 ) ) ;
#59053=CARTESIAN_POINT ( 'NONE',  ( -49.31824139127019180, -278.0374561077733802, -197.0983857279997267 ) ) ;
#59054=CARTESIAN_POINT ( 'NONE',  ( -1.357977749472828455, -280.5748210327720926, -336.1797120751910484 ) ) ;
#59056=CARTESIAN_POINT ( 'NONE',  ( -101.5244020387511341, -276.4845445126429127, -311.7284878036716691 ) ) ;
#59058=CARTESIAN_POINT ( 'NONE',  ( -52.79923344721267853, -299.3707396034314456, -198.2547823274953771 ) ) ;
#59059=CARTESIAN_POINT ( 'NONE',  ( -94.17934335839788673, -282.7700828251171856, -321.8682173719171260 ) ) ;
#59060=CARTESIAN_POINT ( 'NONE',  ( -43.50590004731491689, -274.7752731851270482, -197.4089617291056129 ) ) ;
#59061=CARTESIAN_POINT ( 'NONE',  ( -83.24075413761218556, -274.8628523080236050, -209.2057428890541075 ) ) ;
#59062=CARTESIAN_POINT ( 'NONE',  ( 22.48071900126181433, -275.8036995446516357, -312.3211292519922040 ) ) ;
#59063=CARTESIAN_POINT ( 'NONE',  ( -20.37153152378789400, -296.8344807776048810, -343.4695247431674261 ) ) ;
#59064=CARTESIAN_POINT ( 'NONE',  ( -38.91804670270450117, -289.2380963281947857, -347.3449808111181483 ) ) ;
#59066=CARTESIAN_POINT ( 'NONE',  ( -50.66131443997187489, -277.9631422608254070, -195.9843603897674029 ) ) ;
#59067=CARTESIAN_POINT ( 'NONE',  ( -109.4730951778205394, -290.7279668149149074, -243.2636462022585420 ) ) ;
#59071=CARTESIAN_POINT ( 'NONE',  ( -108.8951816176935097, -289.4049964021939445, -286.0241950955173706 ) ) ;
#59072=CARTESIAN_POINT ( 'NONE',  ( -9.236426670508436132, -290.4194269153589971, -200.8262759705705207 ) ) ;
#59075=CARTESIAN_POINT ( 'NONE',  ( -100.3602033031739609, -289.5514303536575085, -307.4290974135429906 ) ) ;
#59077=CIRCLE ( 'NONE', #54519, 2.186979415864515275 ) ;
#59078=CARTESIAN_POINT ( 'NONE',  ( 29.91959850135221899, -288.0115359480757888, -233.2543962794700292 ) ) ;
#59079=CARTESIAN_POINT ( 'NONE',  ( 27.33386217378599881, -295.6233781216987495, -239.1787733560258573 ) ) ;
#59080=CARTESIAN_POINT ( 'NONE',  ( -0.8286853145115329333, -293.6381952032917866, -337.9009148296640319 ) ) ;
#59081=CARTESIAN_POINT ( 'NONE',  ( 21.24325495529707197, -283.5340859632416937, -319.5658058905803500 ) ) ;
#59083=CARTESIAN_POINT ( 'NONE',  ( -110.3092621230438510, -284.4141758594314524, -268.1851352172002976 ) ) ;
#59084=CARTESIAN_POINT ( 'NONE',  ( 35.86788377100840108, -276.7755592877944650, -263.3572010220200355 ) ) ;
#59085=CARTESIAN_POINT ( 'NONE',  ( 37.35376758639417005, -291.5778394467686780, -270.7940726316613222 ) ) ;
#59086=CARTESIAN_POINT ( 'NONE',  ( -76.76464319899919531, -272.3062727201800044, -208.4501975885578702 ) ) ;
#59088=CARTESIAN_POINT ( 'NONE',  ( -114.4693872376281121, -273.8646567567205921, -270.3778293100139081 ) ) ;
#59089=CARTESIAN_POINT ( 'NONE',  ( -53.28901166602894790, -294.9178646318595725, -345.7245277394727054 ) ) ;
#59090=CARTESIAN_POINT ( 'NONE',  ( -41.42591119986312975, -287.9205116072261603, -196.0204954558087138 ) ) ;
#59091=CARTESIAN_POINT ( 'NONE',  ( -98.85277881934371180, -298.2436921384124275, -224.5365786145442257 ) ) ;
#59093=CARTESIAN_POINT ( 'NONE',  ( 17.84770293480332626, -287.5211043880350417, -222.4234244837805647 ) ) ;
#59094=CARTESIAN_POINT ( 'NONE',  ( -108.4430235737596178, -277.2422597555933521, -299.2993628611334884 ) ) ;
#59095=CARTESIAN_POINT ( 'NONE',  ( -66.87760821092773256, -296.0805633125021927, -341.3748981024409090 ) ) ;
#59096=CARTESIAN_POINT ( 'NONE',  ( 23.14161440105112177, -286.3092921343909438, -315.9908686596827465 ) ) ;
#59097=CARTESIAN_POINT ( 'NONE',  ( 37.40039647763912001, -293.6549142209549927, -251.9393024743903311 ) ) ;
#59098=CARTESIAN_POINT ( 'NONE',  ( -41.59831225575243963, -292.3304886612406222, -197.4142837545906843 ) ) ;
#59101=CARTESIAN_POINT ( 'NONE',  ( 202.9739431815425235, 291.9636489454802017, -68.24819713443925195 ) ) ;
#59102=CARTESIAN_POINT ( 'NONE',  ( 28.09393383406584377, -288.5545145537709004, -231.0051378809324376 ) ) ;
#59103=CARTESIAN_POINT ( 'NONE',  ( -72.08107566293803359, -280.9809262143061233, -342.4248175857292154 ) ) ;
#59105=CARTESIAN_POINT ( 'NONE',  ( -111.6303997534848520, -278.1503381933561059, -250.4482305831111546 ) ) ;
#59106=CARTESIAN_POINT ( 'NONE',  ( 10.42774253480610547, -282.7130705988873274, -212.6905608907666760 ) ) ;
#59107=CARTESIAN_POINT ( 'NONE',  ( 201.1965474191012504, 286.6890272589430424, -96.92993898827639043 ) ) ;
#59108=CARTESIAN_POINT ( 'NONE',  ( -69.52797545116446543, -284.2115517108798599, -201.0457095323620251 ) ) ;
#59109=CARTESIAN_POINT ( 'NONE',  ( 35.09683540725919215, -285.8538167795406935, -287.5067521566995765 ) ) ;
#59110=CARTESIAN_POINT ( 'NONE',  ( -49.54403497918417543, -275.7587145875591546, -195.5324524860870099 ) ) ;
#59111=CARTESIAN_POINT ( 'NONE',  ( -36.48879044673999061, -298.5554612201654550, -197.2995053034559021 ) ) ;
#59113=CARTESIAN_POINT ( 'NONE',  ( 17.43703797275952638, -292.9333689359762047, -319.3753243287773103 ) ) ;
#59114=CARTESIAN_POINT ( 'NONE',  ( -106.2503485270460288, -278.7629663289929454, -304.6116875327993512 ) ) ;
#59115=CARTESIAN_POINT ( 'NONE',  ( 30.27802776076735825, -275.9222054910284783, -298.0014827827318413 ) ) ;
#59116=CARTESIAN_POINT ( 'NONE',  ( -102.4638420214725301, -274.1638313190111944, -229.8568077856197078 ) ) ;
#59117=CARTESIAN_POINT ( 'NONE',  ( -73.96139778352669225, -276.4471866244645071, -337.7592209991657910 ) ) ;
#59118=CARTESIAN_POINT ( 'NONE',  ( -110.5173715819909575, -266.5038384662269095, -306.9164069516367590 ) ) ;
#59119=CARTESIAN_POINT ( 'NONE',  ( 36.28522939467180919, -273.3677241083664740, -256.0098019135094205 ) ) ;
#59120=CARTESIAN_POINT ( 'NONE',  ( -97.79705253300559775, -297.3488111491417953, -317.0918002014356603 ) ) ;
#59123=CARTESIAN_POINT ( 'NONE',  ( -98.37199123406922752, -286.1932347336254452, -229.7467160887507021 ) ) ;
#59124=CARTESIAN_POINT ( 'NONE',  ( -66.17075887807945378, -285.1844665087870112, -340.6805870677355301 ) ) ;
#59125=CARTESIAN_POINT ( 'NONE',  ( -35.92318276719742443, -285.4189953989413198, -197.2729487824906300 ) ) ;
#59126=CARTESIAN_POINT ( 'NONE',  ( -102.8567936818223387, -277.4103837043670069, -236.2762466137838544 ) ) ;
#59127=CARTESIAN_POINT ( 'NONE',  ( -92.56837818269444540, -285.7141611097057421, -319.9874909923241830 ) ) ;
#59128=CARTESIAN_POINT ( 'NONE',  ( -38.34401603073168019, -278.5192435690294701, -196.6620806762900600 ) ) ;
#59129=CARTESIAN_POINT ( 'NONE',  ( 11.96573502319869320, -277.4274542991929025, -324.6794638628950338 ) ) ;
#59131=CARTESIAN_POINT ( 'NONE',  ( -19.26245373214130296, -274.7833328453204444, -199.5193174185405098 ) ) ;
#59132=CARTESIAN_POINT ( 'NONE',  ( 28.17268597888741510, -282.8817997075269659, -310.6119905462495012 ) ) ;
#59133=CARTESIAN_POINT ( 'NONE',  ( -34.47498158608785701, -283.5093668984592910, -347.2461544213545039 ) ) ;
#59137=CARTESIAN_POINT ( 'NONE',  ( 15.42172952163182842, -288.6488663652718287, -215.9890114335678675 ) ) ;
#59138=CARTESIAN_POINT ( 'NONE',  ( -98.79839149250919661, -289.8469253770654177, -224.7719379034734004 ) ) ;
#59140=CARTESIAN_POINT ( 'NONE',  ( -102.6719321324302285, -296.1966716442356642, -237.3156512049067715 ) ) ;
#59141=CARTESIAN_POINT ( 'NONE',  ( -7.222471578065059461, -291.7855478872908179, -199.5926989929982653 ) ) ;
#59142=CARTESIAN_POINT ( 'NONE',  ( -5.510310450117462011, -287.1054780762986525, -336.8251713193008072 ) ) ;
#59143=CARTESIAN_POINT ( 'NONE',  ( -21.01613257656125455, -287.4132519910804717, -342.1166108700935524 ) ) ;
#59144=CARTESIAN_POINT ( 'NONE',  ( -60.11632823701467032, -286.9553389800802279, -200.5868618510524186 ) ) ;
#59145=CARTESIAN_POINT ( 'NONE',  ( -110.4464167217849848, -276.7671167876472964, -253.6069822085198382 ) ) ;
#59146=CARTESIAN_POINT ( 'NONE',  ( 37.57823079558884416, -289.4951776762216582, -265.9110003796409387 ) ) ;
#59147=CARTESIAN_POINT ( 'NONE',  ( -68.61826181696213212, -287.4620365835401117, -338.7258051652080439 ) ) ;
#59148=CIRCLE ( 'NONE', #92367, 2.397123461337413719 ) ;
#59149=CARTESIAN_POINT ( 'NONE',  ( -102.4530433121057627, -285.9476772324411513, -236.8361804557841026 ) ) ;
#59150=CARTESIAN_POINT ( 'NONE',  ( -112.5355219157387552, -292.5770836622889419, -268.4278995277938975 ) ) ;
#59153=CARTESIAN_POINT ( 'NONE',  ( -77.45902287679265896, -299.4385109443612691, -206.3305423765728221 ) ) ;
#59154=CARTESIAN_POINT ( 'NONE',  ( 0.4921901685661741466, -279.7671358742132384, -207.6829960213547963 ) ) ;
#59155=CARTESIAN_POINT ( 'NONE',  ( 25.80085034987899206, -280.0980954989550469, -310.9289899061022879 ) ) ;
#59156=CARTESIAN_POINT ( 'NONE',  ( -5.873200673730681665, -293.8460328441070146, -340.4602789128251743 ) ) ;
#59157=CARTESIAN_POINT ( 'NONE',  ( -36.45111023169724973, -296.4633527993654525, -196.5613598044025139 ) ) ;
#59158=CARTESIAN_POINT ( 'NONE',  ( 14.72132402073479795, -274.3922792783134810, -323.6377286171231162 ) ) ;
#59159=CARTESIAN_POINT ( 'NONE',  ( -0.4963008571692998361, -295.8669956767841995, -334.0089867835717428 ) ) ;
#59161=CARTESIAN_POINT ( 'NONE',  ( -106.8370676071185841, -295.1908193906509155, -239.5005421950999676 ) ) ;
#59162=CARTESIAN_POINT ( 'NONE',  ( -7.734722263637749506, -296.0816355774206272, -337.7454367609204837 ) ) ;
#59164=CARTESIAN_POINT ( 'NONE',  ( -66.10723174152366255, -296.2413803868636251, -337.6303228113463888 ) ) ;
#59165=DIRECTION ( 'NONE',  ( -1.000000000000000000, 0.000000000000000000, -0.000000000000000000 ) ) ;
#59166=CARTESIAN_POINT ( 'NONE',  ( -77.62151472661336982, -283.5343936517504631, -206.6748295253652827 ) ) ;
#59167=CARTESIAN_POINT ( 'NONE',  ( -110.0503104255924427, -296.6453045863960369, -263.2996556057767066 ) ) ;
#59168=CARTESIAN_POINT ( 'NONE',  ( -91.90299058957434397, -285.2994675404841018, -216.0282036195645787 ) ) ;
#59169=CARTESIAN_POINT ( 'NONE',  ( -1.045274000729234931, -284.4945023242057118, -336.6470681121771804 ) ) ;
#59170=CARTESIAN_POINT ( 'NONE',  ( -87.73289502608102453, -285.0376039517623212, -212.0971533066257848 ) ) ;
#59171=CARTESIAN_POINT ( 'NONE',  ( 5.575401975249509867, -290.6342601261230811, -208.9938232435833072 ) ) ;
#59172=CARTESIAN_POINT ( 'NONE',  ( -111.7309490133388010, -277.6559685721651363, -289.8949852356172414 ) ) ;
#59173=CARTESIAN_POINT ( 'NONE',  ( -54.42813229853332757, -277.3380690714490129, -195.3538533559490702 ) ) ;
#59175=CARTESIAN_POINT ( 'NONE',  ( 20.66384458098975330, -285.7170958360764530, -225.3890456588433153 ) ) ;
#59176=CARTESIAN_POINT ( 'NONE',  ( -43.17256257768601557, -288.0444856609815361, -346.8300237736628446 ) ) ;
#59178=CARTESIAN_POINT ( 'NONE',  ( -110.0676516180343754, -298.3159795585962115, -257.8161430496942899 ) ) ;
#59179=CARTESIAN_POINT ( 'NONE',  ( -92.65981265102122677, -280.7042869482132232, -217.5738997647169981 ) ) ;
#59180=CARTESIAN_POINT ( 'NONE',  ( -68.86336441560726485, -293.4845996708365305, -338.8207820590514530 ) ) ;
#59181=CARTESIAN_POINT ( 'NONE',  ( 35.05432814463167546, -281.0881727064717097, -260.4507349593490630 ) ) ;
#59182=CARTESIAN_POINT ( 'NONE',  ( 38.07101924524830849, -293.9133534756608697, -285.9149522766757627 ) ) ;
#59183=CARTESIAN_POINT ( 'NONE',  ( -30.98025349358860225, -284.2117651929289650, -195.0563311550190519 ) ) ;
#59184=CARTESIAN_POINT ( 'NONE',  ( -76.47137807786182861, -281.5293517993033561, -206.3176356285933082 ) ) ;
#59185=CARTESIAN_POINT ( 'NONE',  ( -75.79176179874217212, -294.6375474653270885, -332.7500238143072693 ) ) ;
#59186=CARTESIAN_POINT ( 'NONE',  ( -36.54089470230270820, -296.0620199789775029, -195.3613822856206639 ) ) ;
#59189=CARTESIAN_POINT ( 'NONE',  ( 34.92206208694674530, -283.7740998633518075, -289.1149191388742565 ) ) ;
#59190=CARTESIAN_POINT ( 'NONE',  ( -110.4457867465490892, -296.0453469947829603, -271.4577890013238743 ) ) ;
#59192=CARTESIAN_POINT ( 'NONE',  ( -67.68488546085839630, -295.1237833571632336, -207.2794874003663779 ) ) ;
#59193=CARTESIAN_POINT ( 'NONE',  ( -29.84444656902484638, -273.3419492227055798, -193.8892276605981522 ) ) ;
#59194=CARTESIAN_POINT ( 'NONE',  ( -105.7098950466958058, -290.7285624476944008, -244.6288303902620953 ) ) ;
#59195=CARTESIAN_POINT ( 'NONE',  ( -54.67446553266402276, -281.3456057943258770, -198.6824275501904253 ) ) ;
#59196=CARTESIAN_POINT ( 'NONE',  ( -64.88608884330454885, -275.2864340038062210, -201.8803645821617181 ) ) ;
#59197=CARTESIAN_POINT ( 'NONE',  ( -58.24749520386723134, -284.9179244132961912, -343.6921444374638668 ) ) ;
#59199=CARTESIAN_POINT ( 'NONE',  ( -66.21182856767805447, -278.4605520009587281, -202.8666964932214398 ) ) ;
#59200=CARTESIAN_POINT ( 'NONE',  ( 6.588326621156112672, -278.4556149077121177, -331.2130385379214772 ) ) ;
#59202=CARTESIAN_POINT ( 'NONE',  ( -93.17070340428988118, -273.1103786707471954, -217.3124288204401751 ) ) ;
#59203=CARTESIAN_POINT ( 'NONE',  ( -104.8727395650716829, -292.8868704139201213, -239.0422273977443695 ) ) ;
#59207=CARTESIAN_POINT ( 'NONE',  ( -44.69963521150854291, -293.2837783280903636, -345.8203413287523631 ) ) ;
#59208=CARTESIAN_POINT ( 'NONE',  ( -11.46256119620454506, -273.9060860241622777, -201.9823683891267763 ) ) ;
#59210=CARTESIAN_POINT ( 'NONE',  ( -64.16339541989695761, -293.2287500592112224, -198.8680281018717153 ) ) ;
#59211=CARTESIAN_POINT ( 'NONE',  ( -4.829096099716510437, -276.9805209788416391, -202.7746430608542312 ) ) ;
#59212=CARTESIAN_POINT ( 'NONE',  ( -11.40998174010726807, -288.3909272590983051, -200.1644342461136148 ) ) ;
#59213=CARTESIAN_POINT ( 'NONE',  ( -8.043811174191334956, -274.6673593766132626, -339.2347260110625484 ) ) ;
#59214=CARTESIAN_POINT ( 'NONE',  ( 26.62522777561350296, -277.9855948300413502, -308.4340260761187551 ) ) ;
#59216=CARTESIAN_POINT ( 'NONE',  ( 32.89067710666319755, -291.9557184457170820, -295.1877136296014896 ) ) ;
#59217=CARTESIAN_POINT ( 'NONE',  ( -110.1568037434600313, -280.6793131326099342, -249.4263104331916168 ) ) ;
#59219=CARTESIAN_POINT ( 'NONE',  ( -73.81103255392446272, -283.2171054920654001, -333.6806976298589689 ) ) ;
#59220=CARTESIAN_POINT ( 'NONE',  ( -95.67965454365463529, -280.3061380527026927, -220.5596657276281292 ) ) ;
#59221=CARTESIAN_POINT ( 'NONE',  ( -66.43970661227905339, -282.2197283635438225, -341.2364679255416036 ) ) ;
#59222=CARTESIAN_POINT ( 'NONE',  ( 8.111420726632259104, -277.3891119227836271, -332.2883473100196738 ) ) ;
#59224=CARTESIAN_POINT ( 'NONE',  ( 36.60848089217793699, -276.8346664066436915, -251.5441447462659710 ) ) ;
#59225=CARTESIAN_POINT ( 'NONE',  ( -102.0455923789670294, -287.4805209788416391, -239.2376011013261916 ) ) ;
#59226=ORIENTED_EDGE ( 'NONE', *, *, #23628, .F. ) ;
#59227=ORIENTED_EDGE ( 'NONE', *, *, #22848, .F. ) ;
#59228=CARTESIAN_POINT ( 'NONE',  ( -110.8397082590496439, -298.3597315960658420, -285.3596097409123900 ) ) ;
#59229=CARTESIAN_POINT ( 'NONE',  ( -70.37225221874938086, -292.6857564760307469, -204.9148904125863737 ) ) ;
#59230=CARTESIAN_POINT ( 'NONE',  ( -74.86134914474827440, -275.5744971127168697, -334.8911322453533899 ) ) ;
#59231=CARTESIAN_POINT ( 'NONE',  ( -51.47456847335546826, -290.9906497894075983, -345.0219245932429430 ) ) ;
#59232=CARTESIAN_POINT ( 'NONE',  ( -72.66894332555671099, -290.9201509496366498, -206.3051867135904729 ) ) ;
#59233=CARTESIAN_POINT ( 'NONE',  ( 14.55756891908503725, -287.8528824296484459, -327.2311315124798057 ) ) ;
#59235=CARTESIAN_POINT ( 'NONE',  ( -81.11687103102769925, -282.0575584705125607, -329.8399852014875364 ) ) ;
#59236=CARTESIAN_POINT ( 'NONE',  ( -91.47756380452071312, -291.6930371038618546, -321.2315699822405008 ) ) ;
#59237=CARTESIAN_POINT ( 'NONE',  ( -71.48240004584029350, -284.0724622956608414, -205.0532290022398172 ) ) ;
#59238=CARTESIAN_POINT ( 'NONE',  ( -38.37752109014439128, -281.3540799613490435, -196.8627803948396320 ) ) ;
#59239=CARTESIAN_POINT ( 'NONE',  ( -112.0309622264713738, -291.2702822745546314, -288.1468021035003630 ) ) ;
#59240=CARTESIAN_POINT ( 'NONE',  ( -62.33588742353349232, -280.2105521026131214, -201.6543885923783819 ) ) ;
#59241=CARTESIAN_POINT ( 'NONE',  ( -61.54847960909332016, -290.5395757737460372, -197.6276065480706450 ) ) ;
#59242=CARTESIAN_POINT ( 'NONE',  ( 38.81386786641555631, -288.2268739638572015, -260.1391669055101374 ) ) ;
#59243=CARTESIAN_POINT ( 'NONE',  ( 32.81133645269277821, -288.4483560594792380, -301.9534962019183695 ) ) ;
#59244=CARTESIAN_POINT ( 'NONE',  ( -37.28300403395834905, -286.2195510699564238, -197.3487029993409863 ) ) ;
#59247=CARTESIAN_POINT ( 'NONE',  ( 16.59338243036610905, -294.6691324593296031, -217.0771901050731856 ) ) ;
#59248=CARTESIAN_POINT ( 'NONE',  ( -112.7209512462045780, -295.0684851726238662, -283.7477506012513686 ) ) ;
#59249=CARTESIAN_POINT ( 'NONE',  ( 16.69670121250682726, -275.3178931601833028, -319.8091583717057347 ) ) ;
#59250=CARTESIAN_POINT ( 'NONE',  ( -14.83883542817090806, -297.6755480047640958, -193.4654597526000259 ) ) ;
#59251=CARTESIAN_POINT ( 'NONE',  ( 36.11400074986045183, -292.1092963467750678, -276.2744723384471399 ) ) ;
#59252=CARTESIAN_POINT ( 'NONE',  ( -102.0903711785251460, -295.2753630931429711, -234.5060819548803011 ) ) ;
#59253=CARTESIAN_POINT ( 'NONE',  ( -2.263090077083370399, -293.7323999285008540, -205.8749799484477876 ) ) ;
#59254=CARTESIAN_POINT ( 'NONE',  ( 27.75474069749391504, -294.1752578669907621, -236.6464406962314797 ) ) ;
#59256=CARTESIAN_POINT ( 'NONE',  ( 31.72178143607572309, -291.9406376179620111, -300.1617040198403288 ) ) ;
#59257=CARTESIAN_POINT ( 'NONE',  ( -110.3348684007941074, -298.3303865942214088, -287.6494786358357487 ) ) ;
#59258=CARTESIAN_POINT ( 'NONE',  ( -110.4813975845010816, -291.5542706618424518, -265.7326542436144337 ) ) ;
#59260=CARTESIAN_POINT ( 'NONE',  ( -92.20375653846130604, -296.1977177104774910, -318.5507668010619113 ) ) ;
#59261=EDGE_CURVE ( 'NONE', #1315, #78913, #56242, .T. ) ;
#59262=CARTESIAN_POINT ( 'NONE',  ( -74.50265332788968919, -279.5238568493255116, -335.9162120704741028 ) ) ;
#59263=CARTESIAN_POINT ( 'NONE',  ( -99.83642463930009114, -277.8247399392926695, -226.2282766793475446 ) ) ;
#59265=CARTESIAN_POINT ( 'NONE',  ( -60.83207967364867841, -273.1038588933913616, -197.0831979786206603 ) ) ;
#59266=CARTESIAN_POINT ( 'NONE',  ( -4.207743384126525932, -280.6916773842535804, -337.0203642425162798 ) ) ;
#59267=CARTESIAN_POINT ( 'NONE',  ( -112.9748177434362333, -276.8294893736833728, -280.0572769153680497 ) ) ;
#59268=CARTESIAN_POINT ( 'NONE',  ( -98.73648959464510710, -277.1398640988450097, -226.9939846412351585 ) ) ;
#59269=CARTESIAN_POINT ( 'NONE',  ( -60.65658042419239848, -296.4282212249879080, -200.6103780403647079 ) ) ;
#59270=CARTESIAN_POINT ( 'NONE',  ( -111.1207100805108894, -274.7289146363895611, -256.6068679754121149 ) ) ;
#59272=CARTESIAN_POINT ( 'NONE',  ( 202.9738562182569694, 293.9636489450776367, -54.00000000000000000 ) ) ;
#59274=CARTESIAN_POINT ( 'NONE',  ( -98.67728077941929143, -289.1647727934766294, -226.5849446631862065 ) ) ;
#59275=CARTESIAN_POINT ( 'NONE',  ( -99.02913569081883338, -289.9388116324683438, -316.4661107424431634 ) ) ;
#59276=CARTESIAN_POINT ( 'NONE',  ( -57.65134353210236640, -275.7908285796809764, -197.9361099450058248 ) ) ;
#59277=CARTESIAN_POINT ( 'NONE',  ( -70.03608324650180350, -295.6202805425906490, -203.0476294105857278 ) ) ;
#59278=CARTESIAN_POINT ( 'NONE',  ( -50.07683459419514804, -282.4077383118568605, -346.1907027889089363 ) ) ;
#59281=CARTESIAN_POINT ( 'NONE',  ( -61.07922065363230502, -281.3599954497074691, -341.5596076309277009 ) ) ;
#59283=CARTESIAN_POINT ( 'NONE',  ( 31.20467217984041142, -291.9985318348604437, -244.1213514528446353 ) ) ;
#59284=CARTESIAN_POINT ( 'NONE',  ( -106.7108908541011232, -283.0388164732166274, -243.9266545574677991 ) ) ;
#59286=DIRECTION ( 'NONE',  ( 0.9951408606192334583, 0.000000000000000000, -0.09846150276129006507 ) ) ;
#59287=CARTESIAN_POINT ( 'NONE',  ( 30.55977380720766590, -291.1318313154431507, -238.3889629391739788 ) ) ;
#59288=CARTESIAN_POINT ( 'NONE',  ( -39.15724095186205744, -278.6754442855039429, -344.1387855290308835 ) ) ;
#59289=CARTESIAN_POINT ( 'NONE',  ( -74.07203019836173041, -284.7337305507470546, -337.6429991239047013 ) ) ;
#59290=CARTESIAN_POINT ( 'NONE',  ( 21.64975101761049103, -272.9873163552364872, -223.1248852418183333 ) ) ;
#59291=CARTESIAN_POINT ( 'NONE',  ( -109.4211293791368860, -284.7056479251183418, -258.7253007642735838 ) ) ;
#59292=CARTESIAN_POINT ( 'NONE',  ( 32.66427146491945877, -277.2759605079883158, -293.0445669804720410 ) ) ;
#59293=CARTESIAN_POINT ( 'NONE',  ( 0.9646667953329586265, -277.3299508537898532, -332.7522152491944212 ) ) ;
#59294=CARTESIAN_POINT ( 'NONE',  ( -95.60224190837091385, -285.9016969008304159, -317.6116841705833167 ) ) ;
#59297=CARTESIAN_POINT ( 'NONE',  ( -94.65299584153534340, -295.6875769930560978, -321.8046426537650291 ) ) ;
#59298=CARTESIAN_POINT ( 'NONE',  ( 33.39133284039870375, -289.2222221650000051, -246.5140039186179024 ) ) ;
#59300=CARTESIAN_POINT ( 'NONE',  ( -2.659677404128736544, -286.1237833571631768, -342.4524372437778652 ) ) ;
#59301=CARTESIAN_POINT ( 'NONE',  ( -59.20082964342246612, -278.6959951863848346, -196.8514521837713858 ) ) ;
#59302=CARTESIAN_POINT ( 'NONE',  ( -33.55848996007854623, -290.4989048911011196, -194.2550884100214716 ) ) ;
#59303=CARTESIAN_POINT ( 'NONE',  ( -106.8209977280125855, -285.7466650322019746, -295.0758368735749286 ) ) ;
#59304=CARTESIAN_POINT ( 'NONE',  ( -70.21020943911518941, -281.3731126325400851, -204.0324103728401610 ) ) ;
#59305=CARTESIAN_POINT ( 'NONE',  ( 39.05056830386127587, -288.9562309325569913, -268.6795665767796208 ) ) ;
#59306=CARTESIAN_POINT ( 'NONE',  ( 36.29310367044358543, -283.3685413929187007, -256.0487072342228885 ) ) ;
#59307=CARTESIAN_POINT ( 'NONE',  ( -5.282839820566376687, -276.8084873451835506, -340.3698994339844148 ) ) ;
#59308=CARTESIAN_POINT ( 'NONE',  ( -34.37347169243706446, -296.1095954194135516, -195.7173170109917351 ) ) ;
#59309=CARTESIAN_POINT ( 'NONE',  ( -39.58513240509605424, -279.8580645595582723, -193.3807559228765172 ) ) ;
#59310=CARTESIAN_POINT ( 'NONE',  ( -80.58402723695006387, -299.3808182795068547, -209.7689126954684582 ) ) ;
#59312=CARTESIAN_POINT ( 'NONE',  ( -54.42813229853333468, -279.7662352645560304, -345.3683826091709648 ) ) ;
#59313=CARTESIAN_POINT ( 'NONE',  ( -103.3381623678167216, -271.2889261532651517, -232.5933796212814286 ) ) ;
#59315=CARTESIAN_POINT ( 'NONE',  ( -27.54392032566019566, -279.6874896496641441, -197.9082815646748941 ) ) ;
#59316=CARTESIAN_POINT ( 'NONE',  ( -8.022344194352687197, -277.8816078899575359, -341.1452680859304678 ) ) ;
#59317=CARTESIAN_POINT ( 'NONE',  ( -71.64438704873737152, -282.5530624709564336, -339.0353189897990660 ) ) ;
#59318=CARTESIAN_POINT ( 'NONE',  ( -61.56580197023708223, -291.1313803830333313, -340.2979959691291469 ) ) ;
#59319=CARTESIAN_POINT ( 'NONE',  ( -54.45863097250634866, -299.3562124186790356, -195.9990414290667218 ) ) ;
#59320=CARTESIAN_POINT ( 'NONE',  ( 7.683387436728358111, -299.8091520019872291, -193.7491945106231697 ) ) ;
#59321=CARTESIAN_POINT ( 'NONE',  ( -25.13450700442725605, -294.2081860212998095, -196.4773743154284773 ) ) ;
#59322=CARTESIAN_POINT ( 'NONE',  ( 35.23983971529512615, -279.3168326724843951, -252.0895293219945756 ) ) ;
#59323=CARTESIAN_POINT ( 'NONE',  ( -59.35101031626653167, -285.2593207658308074, -341.5272172051828079 ) ) ;
#59324=CARTESIAN_POINT ( 'NONE',  ( -59.95035027100280445, -271.7779839509131534, -199.1684437841001625 ) ) ;
#59325=CARTESIAN_POINT ( 'NONE',  ( -113.0274302840048790, -286.2639703026810594, -261.5230941430026519 ) ) ;
#59327=CARTESIAN_POINT ( 'NONE',  ( -70.12298574114360861, -288.4148760625993191, -335.9464746435422740 ) ) ;
#59328=CARTESIAN_POINT ( 'NONE',  ( -103.0630025851773865, -256.8465833436261505, -326.7099068919612250 ) ) ;
#59330=CARTESIAN_POINT ( 'NONE',  ( 5.213997448806920509, -287.0633906515332683, -333.8246421162912725 ) ) ;
#59331=CARTESIAN_POINT ( 'NONE',  ( -80.42340096351985324, -289.3206278847395083, -329.3821154119235075 ) ) ;
#59333=CARTESIAN_POINT ( 'NONE',  ( -10.11660708030318823, -287.4789080717545176, -198.6087559490982244 ) ) ;
#59334=CARTESIAN_POINT ( 'NONE',  ( 34.86192568907098632, -275.7406304692809158, -259.3809695100936210 ) ) ;
#59335=CARTESIAN_POINT ( 'NONE',  ( 35.16489085092543831, -292.1544512647576539, -245.2145508401879113 ) ) ;
#59336=CARTESIAN_POINT ( 'NONE',  ( 36.38333763275200994, -282.4802768894000451, -292.4060171876651566 ) ) ;
#59337=CARTESIAN_POINT ( 'NONE',  ( 36.87856427347627175, -283.2965720612031646, -288.1386546930356189 ) ) ;
#59338=CARTESIAN_POINT ( 'NONE',  ( -61.22108016712463296, -283.6870853797404948, -343.5982009010909337 ) ) ;
#59339=CARTESIAN_POINT ( 'NONE',  ( 15.27167089700801483, -281.1538305122716110, -219.6537169291917451 ) ) ;
#59340=CARTESIAN_POINT ( 'NONE',  ( -105.5937364680635966, -293.8380690714490129, -285.9065529553535612 ) ) ;
#59341=CARTESIAN_POINT ( 'NONE',  ( -63.41909885852727058, -182.9725237402124947, -362.5579290312759895 ) ) ;
#59344=CARTESIAN_POINT ( 'NONE',  ( -88.32644975019017863, -279.7686299980030071, -325.1387021782032321 ) ) ;
#59345=CARTESIAN_POINT ( 'NONE',  ( 196.7050999029026741, 285.3698064150070195, -111.6815863925781116 ) ) ;
#59347=CARTESIAN_POINT ( 'NONE',  ( -109.9067179730154322, -295.7788906872280563, -279.6105235613302398 ) ) ;
#59348=CARTESIAN_POINT ( 'NONE',  ( 39.16563853981011789, -292.9518892385784739, -261.7390483411336959 ) ) ;
#59349=CARTESIAN_POINT ( 'NONE',  ( 26.24832809216016116, -24.45034260803730675, -341.6199306126845272 ) ) ;
#59351=CARTESIAN_POINT ( 'NONE',  ( -109.6303901606406157, -271.5548738973836294, -245.3083024605653577 ) ) ;
#59352=CARTESIAN_POINT ( 'NONE',  ( -29.10383471639088881, -287.3458804985839379, -343.6999070914222898 ) ) ;
#59353=CARTESIAN_POINT ( 'NONE',  ( -108.0384440827360919, -298.1152945166665518, -293.1732387303364931 ) ) ;
#59354=CARTESIAN_POINT ( 'NONE',  ( -44.08619489208993514, -287.2802689358219368, -197.1780921612973145 ) ) ;
#59356=CARTESIAN_POINT ( 'NONE',  ( -74.48198181312594102, -296.4745945953837918, -337.6026333411576275 ) ) ;
#59358=CARTESIAN_POINT ( 'NONE',  ( -49.43788583444410989, -286.3862593689379423, -198.2563260900890612 ) ) ;
#59359=CARTESIAN_POINT ( 'NONE',  ( -106.1498907570397989, -295.7816561999024998, -236.6944932656572576 ) ) ;
#59360=CARTESIAN_POINT ( 'NONE',  ( 24.67806120022697414, -293.7514493957186232, -224.9991512524795212 ) ) ;
#59361=CARTESIAN_POINT ( 'NONE',  ( 38.79006878958215765, -293.9009414740083912, -258.8916612788188445 ) ) ;
#59362=CARTESIAN_POINT ( 'NONE',  ( -102.4105294853175110, -291.1696053634590839, -237.1577128703661401 ) ) ;
#59365=CARTESIAN_POINT ( 'NONE',  ( -91.16087824626904990, -275.2146166960715732, -217.3251842788459953 ) ) ;
#59366=CARTESIAN_POINT ( 'NONE',  ( -7.829295294427161878, -273.2251692674003607, -199.6151562959837804 ) ) ;
#59368=CARTESIAN_POINT ( 'NONE',  ( -28.61424944481396082, -276.4520750048379796, -346.8565137576001121 ) ) ;
#59369=CARTESIAN_POINT ( 'NONE',  ( -101.4021778827159750, -271.4498995545723687, -233.6155905375105135 ) ) ;
#59370=CARTESIAN_POINT ( 'NONE',  ( -109.4957424123521719, -280.6390270605056685, -252.9066152519873754 ) ) ;
#59371=CARTESIAN_POINT ( 'NONE',  ( 6.100763367172952201, -274.5956598465853062, -330.6210762945250394 ) ) ;
#59372=CARTESIAN_POINT ( 'NONE',  ( -79.04215355750585559, -274.5550213912567870, -210.0060134684726734 ) ) ;
#59373=CARTESIAN_POINT ( 'NONE',  ( -87.50316644905679198, -274.2729004289537897, -216.9321784089285927 ) ) ;
#59374=CARTESIAN_POINT ( 'NONE',  ( -96.16606327408037203, -274.9668513061713497, -222.2402007114817195 ) ) ;
#59375=CARTESIAN_POINT ( 'NONE',  ( -89.01620676094657370, -271.3506796356424502, -215.4432606239321046 ) ) ;
#59376=CARTESIAN_POINT ( 'NONE',  ( -20.81707905155414551, -295.4859505330491061, -341.6230544575838053 ) ) ;
#59377=CARTESIAN_POINT ( 'NONE',  ( 36.01032612811046363, -292.2041307392824478, -276.2649438748000534 ) ) ;
#59379=CARTESIAN_POINT ( 'NONE',  ( -84.82347076495847205, -278.1790308836919507, -330.9681225577662076 ) ) ;
#59381=CARTESIAN_POINT ( 'NONE',  ( 9.483454273817326197, -274.8834623247841478, -214.2913085253646273 ) ) ;
#59382=CARTESIAN_POINT ( 'NONE',  ( -109.7632989416309215, -282.9242008817736860, -295.0270924731030391 ) ) ;
#59383=CARTESIAN_POINT ( 'NONE',  ( -111.8321738028380139, -298.4185626551264363, -280.8010832467707587 ) ) ;
#59385=CARTESIAN_POINT ( 'NONE',  ( -49.43818209431198341, -285.0912880699073071, -198.1549721843069563 ) ) ;
#59386=CARTESIAN_POINT ( 'NONE',  ( -75.84130907448532355, -281.5643120534360833, -334.9800432270934039 ) ) ;
#59387=CARTESIAN_POINT ( 'NONE',  ( -95.25983415955553824, -276.1499783695610972, -316.4624256863126561 ) ) ;
#59388=CARTESIAN_POINT ( 'NONE',  ( -39.19061369774771464, -275.6505329688265533, -343.9271185348336530 ) ) ;
#59389=CARTESIAN_POINT ( 'NONE',  ( -74.50844179344917961, -281.5579757296370644, -205.2033703588862750 ) ) ;
#59390=CARTESIAN_POINT ( 'NONE',  ( 35.75082462417807960, -276.8448686515374106, -277.0404390222568622 ) ) ;
#59392=CARTESIAN_POINT ( 'NONE',  ( 23.01182561612909439, -273.3244948249692925, -223.8222162592490747 ) ) ;
#59393=CARTESIAN_POINT ( 'NONE',  ( 7.433536390348085554, -282.6608750066078528, -209.9208858560567421 ) ) ;
#59395=CARTESIAN_POINT ( 'NONE',  ( -21.31371410187765747, -288.1763352625901575, -196.5206286891323657 ) ) ;
#59397=CARTESIAN_POINT ( 'NONE',  ( -109.9848977622940822, -288.3117371638712712, -289.0657481500286394 ) ) ;
#59398=CARTESIAN_POINT ( 'NONE',  ( 104.1717476309105166, -299.5541904835127980, -192.9651424135224715 ) ) ;
#59399=CARTESIAN_POINT ( 'NONE',  ( -66.96560624799985817, -296.4499545823885001, -203.1941472263000037 ) ) ;
#59400=CARTESIAN_POINT ( 'NONE',  ( -68.29498457575172665, -289.7807955726265163, -202.8730130505828981 ) ) ;
#59401=CARTESIAN_POINT ( 'NONE',  ( 181.0595704366054690, 252.2700355933461651, -164.3583243123303532 ) ) ;
#59403=CARTESIAN_POINT ( 'NONE',  ( 28.29739534131069334, -286.5436382617302797, -309.2740579564660379 ) ) ;
#59404=CARTESIAN_POINT ( 'NONE',  ( -56.50723799855340701, -284.9034545936958125, -341.6290811309229412 ) ) ;
#59405=CARTESIAN_POINT ( 'NONE',  ( -96.77363491790653427, -283.4344158946931316, -223.0132653902421680 ) ) ;
#59406=CARTESIAN_POINT ( 'NONE',  ( -55.01235538456789698, -291.8185185253624354, -199.5321130283295474 ) ) ;
#59407=CARTESIAN_POINT ( 'NONE',  ( 21.79171467867494627, -282.3679249526834951, -226.5379279028655901 ) ) ;
#59408=CARTESIAN_POINT ( 'NONE',  ( 34.22100641308983171, -282.1540124790445248, -255.0902615840891485 ) ) ;
#59409=CARTESIAN_POINT ( 'NONE',  ( -20.83168193446944017, -290.8212955227522230, -343.9389450386367457 ) ) ;
#59411=CARTESIAN_POINT ( 'NONE',  ( -111.7989246941215242, -273.1324427340867942, -250.6156770818635096 ) ) ;
#59413=CARTESIAN_POINT ( 'NONE',  ( -10.10563266378761504, -286.7791811971883362, -340.8416885479788334 ) ) ;
#59414=CARTESIAN_POINT ( 'NONE',  ( 38.21874907175163116, -275.3668134746865235, -255.5415863867415283 ) ) ;
#59415=CARTESIAN_POINT ( 'NONE',  ( -63.39798318223426321, -293.6908444651630248, -200.4117297377376588 ) ) ;
#59417=CARTESIAN_POINT ( 'NONE',  ( -114.2704648735229114, -281.0519495502701943, -270.3937649182068981 ) ) ;
#59419=CARTESIAN_POINT ( 'NONE',  ( -95.64882087972777924, -275.8997473816919523, -317.8186939487128484 ) ) ;
#59422=CARTESIAN_POINT ( 'NONE',  ( -37.58444860191104908, -296.4490387548829062, -194.1615018943762152 ) ) ;
#59423=CARTESIAN_POINT ( 'NONE',  ( 21.56824034799850054, -274.2951488592610190, -227.0770379815169235 ) ) ;
#59425=CARTESIAN_POINT ( 'NONE',  ( -93.98506786433267735, -292.7349535946738115, -223.2008064314894966 ) ) ;
#59427=CARTESIAN_POINT ( 'NONE',  ( -103.7747757442157024, -291.9081258858419119, -239.5381571974824624 ) ) ;
#59428=CARTESIAN_POINT ( 'NONE',  ( -95.06137381201850189, -285.6663020936589987, -316.7106706680724528 ) ) ;
#59429=CARTESIAN_POINT ( 'NONE',  ( -16.80257704382437822, -293.7376704602239670, -196.7625397737684807 ) ) ;
#59430=CARTESIAN_POINT ( 'NONE',  ( 21.81721147078295076, -294.2116305041512874, -221.8480119889270270 ) ) ;
#59431=CARTESIAN_POINT ( 'NONE',  ( 34.83764836775974061, -293.5337975443893583, -281.6050554926152927 ) ) ;
#59432=CARTESIAN_POINT ( 'NONE',  ( 31.26459995428608352, -289.9507104240859121, -300.7914908447457947 ) ) ;
#59433=CARTESIAN_POINT ( 'NONE',  ( 39.18252616323609772, -281.6061084499941671, -261.3478582940723527 ) ) ;
#59434=CARTESIAN_POINT ( 'NONE',  ( -48.72838308939262930, -295.9882174061281717, -195.6113508563573191 ) ) ;
#59435=CARTESIAN_POINT ( 'NONE',  ( -113.5996787024089940, -284.2473939294193883, -281.4017867208951884 ) ) ;
#59436=CARTESIAN_POINT ( 'NONE',  ( 26.67372381193292341, -277.0144087605440859, -231.8700111909702457 ) ) ;
#59437=CARTESIAN_POINT ( 'NONE',  ( -39.97286786938623493, -284.8132791601767622, -197.0112204908242859 ) ) ;
#59438=CARTESIAN_POINT ( 'NONE',  ( 22.28724812464620442, -284.9291229503145360, -224.8495131303380106 ) ) ;
#59439=CARTESIAN_POINT ( 'NONE',  ( -111.7781241848990561, -276.8721574554319318, -256.1665410827072265 ) ) ;
#59440=CARTESIAN_POINT ( 'NONE',  ( 163.5244876965996923, 234.8495348041943487, -191.6304063886470317 ) ) ;
#59441=CARTESIAN_POINT ( 'NONE',  ( -107.0464464074657229, -283.7698934295147524, -292.2525954982224334 ) ) ;
#59442=CARTESIAN_POINT ( 'NONE',  ( 33.20626902981570083, -283.1406163705468089, -300.3461481427333410 ) ) ;
#59443=CARTESIAN_POINT ( 'NONE',  ( -97.98113466564090857, -288.9803757194330842, -317.4321195966422806 ) ) ;
#59444=CARTESIAN_POINT ( 'NONE',  ( -38.51202282107968955, -278.6667189247613123, -346.5521329573720664 ) ) ;
#59445=CARTESIAN_POINT ( 'NONE',  ( 3.254116427783104726, -277.8343752899252763, -335.2716025056482749 ) ) ;
#59446=CARTESIAN_POINT ( 'NONE',  ( -38.35172133784325155, -279.8724661127399713, -197.3557049113782966 ) ) ;
#59447=CARTESIAN_POINT ( 'NONE',  ( -69.00266535042828764, -275.6136816638878599, -202.7495500415424203 ) ) ;
#59448=CARTESIAN_POINT ( 'NONE',  ( -113.3907224302259351, -292.2128699707654960, -265.5666815589217435 ) ) ;
#59450=CARTESIAN_POINT ( 'NONE',  ( -38.36032238474562917, -293.9855441888782366, -343.6631539932238297 ) ) ;
#59452=CARTESIAN_POINT ( 'NONE',  ( -7.983701101779252518, -294.3233663998176439, -337.2342186125437706 ) ) ;
#59453=CARTESIAN_POINT ( 'NONE',  ( -112.8265981925139698, -291.4607813343548059, -283.9822746103509417 ) ) ;
#59454=CARTESIAN_POINT ( 'NONE',  ( -24.86714133654969316, -280.8669230423494128, -198.3314154228249606 ) ) ;
#59455=CARTESIAN_POINT ( 'NONE',  ( -85.65083665714618633, -272.4608488318901891, -210.7033645879270125 ) ) ;
#59456=CARTESIAN_POINT ( 'NONE',  ( 35.74954845533157766, -287.9006080393311322, -246.2956489235986339 ) ) ;
#59457=CARTESIAN_POINT ( 'NONE',  ( -9.566999919184999257, -289.0322528267125222, -342.1546435947208238 ) ) ;
#59458=CARTESIAN_POINT ( 'NONE',  ( -57.40426851425257126, -286.1193949603739952, -200.0975146608287503 ) ) ;
#59459=CYLINDRICAL_SURFACE ( 'NONE', #38380, 1.895975569037589015 ) ;
#59460=CARTESIAN_POINT ( 'NONE',  ( -110.3856735362975741, -264.4859968940625095, -306.0548468009229168 ) ) ;
#59461=CARTESIAN_POINT ( 'NONE',  ( -55.39694311004227956, -169.5609126108696501, -360.5716228430129604 ) ) ;
#59462=CARTESIAN_POINT ( 'NONE',  ( -54.00061198648864291, -276.4685664602649240, -341.6529881661105605 ) ) ;
#59463=CARTESIAN_POINT ( 'NONE',  ( -94.70346862234369212, -276.8303379994504780, -316.0304190598139371 ) ) ;
#59464=CARTESIAN_POINT ( 'NONE',  ( -105.5882314637777171, -272.6796843899326177, -234.6347546966848654 ) ) ;
#59465=CARTESIAN_POINT ( 'NONE',  ( -37.61793092032886676, -140.8427143539732924, -362.0657075832283454 ) ) ;
#59466=CARTESIAN_POINT ( 'NONE',  ( -37.14515683742537533, -275.7345374253613386, -346.8806914234819487 ) ) ;
#59467=CARTESIAN_POINT ( 'NONE',  ( -61.25117269039499490, -297.1184331212925827, -342.5431654630265257 ) ) ;
#59468=CARTESIAN_POINT ( 'NONE',  ( -77.29404590694403510, -291.9926306616621901, -209.1908759662587727 ) ) ;
#59469=CARTESIAN_POINT ( 'NONE',  ( -75.70816543095332918, -298.3568837329264625, -203.7254810194878019 ) ) ;
#59470=CARTESIAN_POINT ( 'NONE',  ( -48.14994351211366563, -287.8772227586073313, -343.1065388092864055 ) ) ;
#59471=CARTESIAN_POINT ( 'NONE',  ( -81.19906796063573040, -274.1250001016468900, -207.1313751103526215 ) ) ;
#59472=CARTESIAN_POINT ( 'NONE',  ( -95.29036390310834292, -297.3436202330551055, -225.9453400958412033 ) ) ;
#59475=CARTESIAN_POINT ( 'NONE',  ( -87.98476698147007369, -281.2704282057558771, -214.2844385576136688 ) ) ;
#59478=CARTESIAN_POINT ( 'NONE',  ( -13.44700422291602848, -282.2576332801950230, -343.4950390501155084 ) ) ;
#59481=CARTESIAN_POINT ( 'NONE',  ( -101.0873446707604444, -280.1255602741742905, -234.1572663263705181 ) ) ;
#59482=CARTESIAN_POINT ( 'NONE',  ( -112.7149554263138782, -280.4394902463442918, -260.3242335047801816 ) ) ;
#59483=CARTESIAN_POINT ( 'NONE',  ( -57.02838620769510669, -272.2735827212886761, -199.2928208727300614 ) ) ;
#59484=DIRECTION ( 'NONE',  ( 0.000000000000000000, 0.000000000000000000, 1.000000000000000000 ) ) ;
#59486=CARTESIAN_POINT ( 'NONE',  ( -14.31088965566074478, -280.5258175663214502, -201.0358828618031453 ) ) ;
#59488=CARTESIAN_POINT ( 'NONE',  ( 39.46917076413583203, -276.3291498178131746, -268.2998240233352476 ) ) ;
#59489=CARTESIAN_POINT ( 'NONE',  ( 36.74780484157432880, -277.4016548818336787, -258.6275084797254635 ) ) ;
#59490=CARTESIAN_POINT ( 'NONE',  ( -72.58517864369669326, -276.0841571366627250, -338.1732291633564387 ) ) ;
#59493=CARTESIAN_POINT ( 'NONE',  ( 36.53804865116615019, -283.7216709875748393, -285.1999025138948696 ) ) ;
#59495=CARTESIAN_POINT ( 'NONE',  ( -17.37873647507503350, -291.5134670732281279, -199.9231682902452576 ) ) ;
#59497=CARTESIAN_POINT ( 'NONE',  ( 23.78546316888671086, -286.2776520295481077, -223.6835217691885305 ) ) ;
#59498=CARTESIAN_POINT ( 'NONE',  ( -93.34031160941609073, -282.1117546277640713, -318.7759647947202097 ) ) ;
#59499=CARTESIAN_POINT ( 'NONE',  ( -66.81207807889211381, -282.0207516297173242, -337.8052960318701707 ) ) ;
#59500=CARTESIAN_POINT ( 'NONE',  ( 5.140561975330038891, -281.8462486122599557, -210.5080653418146710 ) ) ;
#59501=CARTESIAN_POINT ( 'NONE',  ( -96.22655637268795203, -271.1898637074183398, -223.9114209064198917 ) ) ;
#59503=CARTESIAN_POINT ( 'NONE',  ( 22.75923767732920311, -280.5846590842179467, -317.2257417157809414 ) ) ;
#59504=CARTESIAN_POINT ( 'NONE',  ( 36.39574039698510433, -295.7291575815638680, -284.1343034324547148 ) ) ;
#59506=CARTESIAN_POINT ( 'NONE',  ( -93.67929177431585686, -278.5438956382691345, -316.9636477778738026 ) ) ;
#59507=CARTESIAN_POINT ( 'NONE',  ( -21.39826594332415510, -288.2563288105177435, -196.9047681559327430 ) ) ;
#59509=CARTESIAN_POINT ( 'NONE',  ( -72.78039021578420886, -293.5067239843279481, -203.6125944749465475 ) ) ;
#59511=CARTESIAN_POINT ( 'NONE',  ( 37.37295766519621054, -273.4607588509501284, -263.2559345594654587 ) ) ;
#59512=CARTESIAN_POINT ( 'NONE',  ( -29.00488113929756651, -288.1463427626158023, -346.7994529033159097 ) ) ;
#59513=CARTESIAN_POINT ( 'NONE',  ( 34.55015722702925274, -292.1702439063636803, -287.0900927647830940 ) ) ;
#59515=CARTESIAN_POINT ( 'NONE',  ( -103.5827141873963200, -276.8077934971782952, -302.3124250561784265 ) ) ;
#59516=CARTESIAN_POINT ( 'NONE',  ( -108.6391984751745952, -294.9606741339634937, -249.6842659269705393 ) ) ;
#59517=CARTESIAN_POINT ( 'NONE',  ( -98.51191275177444595, -291.3053432458011116, -311.1203508074016213 ) ) ;
#59520=CARTESIAN_POINT ( 'NONE',  ( 38.96342398434819643, -291.9956997548592881, -267.4822475280382719 ) ) ;
#59521=CARTESIAN_POINT ( 'NONE',  ( 9.522980761087149304, -288.3094352266235774, -213.3511004577532617 ) ) ;
#59522=CARTESIAN_POINT ( 'NONE',  ( -113.3764067926420012, -288.7814431443119361, -271.1949678090483076 ) ) ;
#59523=CARTESIAN_POINT ( 'NONE',  ( 30.49797330927253114, -288.5962818300487811, -241.7133830080311441 ) ) ;
#59525=CARTESIAN_POINT ( 'NONE',  ( 33.86059420307253731, -288.5763625844373337, -287.1788172759117401 ) ) ;
#59526=CARTESIAN_POINT ( 'NONE',  ( 23.57190624233257736, -296.1338818609468717, -314.7443253490573625 ) ) ;
#59528=CARTESIAN_POINT ( 'NONE',  ( 25.53462351905800531, -289.3394627294273391, -314.2080938520719542 ) ) ;
#59529=CARTESIAN_POINT ( 'NONE',  ( -12.03741097901147228, -278.3998112347296683, -199.3267510031387246 ) ) ;
#59530=CARTESIAN_POINT ( 'NONE',  ( -113.0440607827452340, -278.7098822041110111, -284.3940660114665206 ) ) ;
#59531=CARTESIAN_POINT ( 'NONE',  ( -25.39468663578752228, -279.8671760083025788, -194.3149927685418845 ) ) ;
#59532=CARTESIAN_POINT ( 'NONE',  ( -63.68298239005284955, -299.6871102796877722, -200.4638615808408986 ) ) ;
#59533=CARTESIAN_POINT ( 'NONE',  ( -52.46808131195603409, -283.8582324836573889, -196.9023320003765605 ) ) ;
#59534=CARTESIAN_POINT ( 'NONE',  ( -4.999294894772630116, -278.6221756922370218, -203.5417023324997103 ) ) ;
#59535=CARTESIAN_POINT ( 'NONE',  ( -65.84050210953581939, -281.4247720128125252, -339.7494210890263844 ) ) ;
#59536=DIRECTION ( 'NONE',  ( 0.000000000000000000, -1.000000000000000000, 0.000000000000000000 ) ) ;
#59537=CARTESIAN_POINT ( 'NONE',  ( -4.312632069130462931, -275.1045868853428829, -339.1634802805279492 ) ) ;
#59538=CARTESIAN_POINT ( 'NONE',  ( -99.03854656822382196, -298.6266176146861540, -229.9672887946356923 ) ) ;
#59539=CARTESIAN_POINT ( 'NONE',  ( -103.7658233028419943, -283.9740159266211208, -231.9237240757769882 ) ) ;
#59540=CARTESIAN_POINT ( 'NONE',  ( -110.0365319254666474, -297.3712991017988543, -279.6475332947033507 ) ) ;
#59541=CARTESIAN_POINT ( 'NONE',  ( -109.5510143678241661, -274.2948784320151958, -245.3726960788743554 ) ) ;
#59542=CARTESIAN_POINT ( 'NONE',  ( 34.39506666860962270, -275.0390484499698118, -256.7257310647820532 ) ) ;
#59543=CARTESIAN_POINT ( 'NONE',  ( 34.67764176685086142, -295.8223644810156543, -291.3409195127969724 ) ) ;
#59544=CARTESIAN_POINT ( 'NONE',  ( -46.02366285445285854, -289.3259079535359319, -346.9232214442576492 ) ) ;
#59546=CARTESIAN_POINT ( 'NONE',  ( -45.10071797862819665, -278.0346057849507702, -195.1485453294131105 ) ) ;
#59547=CARTESIAN_POINT ( 'NONE',  ( -112.2631837131080204, -290.1625297421371670, -288.1874955572000658 ) ) ;
#59548=CARTESIAN_POINT ( 'NONE',  ( -95.14365093139960550, -288.9791361269830077, -315.3518507413093630 ) ) ;
#59549=CARTESIAN_POINT ( 'NONE',  ( 20.67867814619486921, -290.8968325289162067, -222.8360050655022064 ) ) ;
#59553=CARTESIAN_POINT ( 'NONE',  ( -90.79993995701471476, -290.7754789528456172, -220.5409652362462509 ) ) ;
#59555=CARTESIAN_POINT ( 'NONE',  ( -70.97399007099811286, -286.5604040062812032, -201.3561233273001676 ) ) ;
#59556=CARTESIAN_POINT ( 'NONE',  ( -37.30987171927208124, -291.5519495502701375, -340.3611179825599606 ) ) ;
#59557=CARTESIAN_POINT ( 'NONE',  ( -24.95762099636236542, -293.9567857813126466, -346.1742066921028140 ) ) ;
#59558=CARTESIAN_POINT ( 'NONE',  ( -4.361154404988054623, -283.9417094352826325, -339.4087101677097849 ) ) ;
#59559=CARTESIAN_POINT ( 'NONE',  ( -42.67201101160323162, -285.8163836908742041, -197.5433566314246150 ) ) ;
#59561=CARTESIAN_POINT ( 'NONE',  ( 19.57407412826109550, -277.5214164666213037, -316.8765257896781691 ) ) ;
#59562=CARTESIAN_POINT ( 'NONE',  ( 5.467118782381859887, -290.6545251542821688, -209.1483195387613705 ) ) ;
#59563=CARTESIAN_POINT ( 'NONE',  ( 29.45374299348132752, -273.9376712199444910, -239.8160946851348854 ) ) ;
#59565=CARTESIAN_POINT ( 'NONE',  ( 64.33209501061345748, 48.33985520751024723, -319.1928417150128325 ) ) ;
#59566=CARTESIAN_POINT ( 'NONE',  ( 38.58472444734961471, -293.3785646829250027, -283.1264778917486638 ) ) ;
#59567=CARTESIAN_POINT ( 'NONE',  ( 9.926391277329841500, -288.6294093956313418, -212.8542337877264572 ) ) ;
#59569=CARTESIAN_POINT ( 'NONE',  ( -111.6656575168238561, -297.3936883340443842, -289.3202284930042083 ) ) ;
#59570=CARTESIAN_POINT ( 'NONE',  ( -27.83149326644779009, -286.8275296328849890, -197.8804403266230736 ) ) ;
#59571=CARTESIAN_POINT ( 'NONE',  ( -97.75118954863651766, -276.9757929905859442, -317.7268630104115346 ) ) ;
#59572=CARTESIAN_POINT ( 'NONE',  ( -37.80275380179691780, -292.6979288421708816, -193.4644326399993872 ) ) ;
#59573=CARTESIAN_POINT ( 'NONE',  ( 37.86147189221529885, -285.8141243052073719, -279.9900887539664041 ) ) ;
#59574=CARTESIAN_POINT ( 'NONE',  ( 35.43123181833192348, -293.5671761096620003, -245.1030844619403410 ) ) ;
#59575=CARTESIAN_POINT ( 'NONE',  ( -92.57527218274242387, -291.5658159659975581, -222.5977428409451875 ) ) ;
#59577=CARTESIAN_POINT ( 'NONE',  ( 6.586641810406439035, -59.71310429714220191, -351.1713004201388912 ) ) ;
#59578=CARTESIAN_POINT ( 'NONE',  ( -52.05869819227491035, -287.3873292957083549, -195.4332025923267793 ) ) ;
#59579=CARTESIAN_POINT ( 'NONE',  ( 40.64545035920995986, -279.2666405000204009, -288.1938231032136741 ) ) ;
#59581=CARTESIAN_POINT ( 'NONE',  ( -32.13742060190021022, -281.9052862106516386, -343.4852695911754381 ) ) ;
#59582=CARTESIAN_POINT ( 'NONE',  ( -112.4647011951343103, -278.0086935366750822, -287.1622787266808245 ) ) ;
#59583=CARTESIAN_POINT ( 'NONE',  ( 37.25882013447047569, -283.6362855136566736, -276.8862712139290920 ) ) ;
#59584=CARTESIAN_POINT ( 'NONE',  ( -104.8949806941793241, -262.6824176341613679, -316.8076958637401503 ) ) ;
#59585=CARTESIAN_POINT ( 'NONE',  ( 17.39144175509819235, -280.8642827599528005, -323.7554559144114137 ) ) ;
#59586=CARTESIAN_POINT ( 'NONE',  ( 36.62953843811489207, -285.4382983292776998, -259.9775103678533128 ) ) ;
#59587=CARTESIAN_POINT ( 'NONE',  ( -13.47441790030156383, -276.2192317023518626, -198.4538282407935128 ) ) ;
#59589=CARTESIAN_POINT ( 'NONE',  ( -106.7672262728909658, -297.3482445783442927, -247.4392095802336371 ) ) ;
#59590=CARTESIAN_POINT ( 'NONE',  ( -45.15973353199539986, -293.8379123854019781, -343.4880732176315519 ) ) ;
#59591=CARTESIAN_POINT ( 'NONE',  ( -96.97008280569878025, -278.5508914317156268, -318.9385967114022833 ) ) ;
#59592=CARTESIAN_POINT ( 'NONE',  ( -53.95392964931998847, -277.2712698710034260, -341.4979535680965910 ) ) ;
#59593=CARTESIAN_POINT ( 'NONE',  ( -30.52263579593893184, -299.0768152995971718, -193.5953506817569689 ) ) ;
#59594=CARTESIAN_POINT ( 'NONE',  ( -93.11866633401946558, -276.7502436622364712, -323.0721407381615222 ) ) ;
#59595=CARTESIAN_POINT ( 'NONE',  ( 64.47034098748159181, 48.08436262803363093, -318.7852478019347586 ) ) ;
#59596=CARTESIAN_POINT ( 'NONE',  ( -100.5444961975137090, -276.0073132200173518, -310.8344157179166132 ) ) ;
#59597=CARTESIAN_POINT ( 'NONE',  ( -69.26508263984791824, -296.8892132442754814, -339.7980859590122122 ) ) ;
#59600=CARTESIAN_POINT ( 'NONE',  ( 202.9738562182569694, 291.4636489450776367, -54.00000000000002132 ) ) ;
#59601=CARTESIAN_POINT ( 'NONE',  ( -45.66094997524324839, -284.2396056453231381, -343.2478691523747898 ) ) ;
#59602=CARTESIAN_POINT ( 'NONE',  ( -64.86398251714732055, -285.1668500991312385, -341.2023734020253301 ) ) ;
#59603=CARTESIAN_POINT ( 'NONE',  ( -33.22463155806325119, -285.4538055576810507, -197.3253230840812478 ) ) ;
#59604=CARTESIAN_POINT ( 'NONE',  ( -110.4109710795806762, -277.0918160819856553, -259.6475732372405787 ) ) ;
#59605=CARTESIAN_POINT ( 'NONE',  ( -91.62885509584685906, -285.6964860873844145, -320.9948052486842016 ) ) ;
#59606=CARTESIAN_POINT ( 'NONE',  ( -103.9886997496694789, -277.4543646077049175, -238.7946984259076828 ) ) ;
#59607=CARTESIAN_POINT ( 'NONE',  ( -6.132596549257987917, -277.7117928338157640, -336.7090847301910799 ) ) ;
#59609=CARTESIAN_POINT ( 'NONE',  ( -83.23410202314381934, -273.8959120811493335, -213.5115279246107605 ) ) ;
#59610=CARTESIAN_POINT ( 'NONE',  ( 39.47876753147257745, -282.3135376910310583, -267.0541075799198438 ) ) ;
#59611=CARTESIAN_POINT ( 'NONE',  ( 39.57885165322228715, -282.0031022786512267, -267.0537634741796182 ) ) ;
#59613=ORIENTED_EDGE ( 'NONE', *, *, #76301, .F. ) ;
#59615=CARTESIAN_POINT ( 'NONE',  ( 37.33530907281996747, -289.2489994240452233, -257.4923651067630885 ) ) ;
#59616=CARTESIAN_POINT ( 'NONE',  ( -92.86028351398626057, -296.4263118160515660, -222.6943057946793090 ) ) ;
#59619=CARTESIAN_POINT ( 'NONE',  ( -5.920985965978887933, -291.8030217340574382, -200.1610121239084776 ) ) ;
#59620=CARTESIAN_POINT ( 'NONE',  ( 32.96934510270195773, -286.3237795774564347, -292.6003530207044605 ) ) ;
#59621=CARTESIAN_POINT ( 'NONE',  ( 12.54199498510939570, -286.9156327562212709, -324.5320253765555094 ) ) ;
#59622=CARTESIAN_POINT ( 'NONE',  ( -14.51284509537617495, -290.5920326445378805, -199.9564491749622448 ) ) ;
#59623=CARTESIAN_POINT ( 'NONE',  ( -17.07689196913042196, -287.5246230339130307, -199.7639001854538492 ) ) ;
#59624=CARTESIAN_POINT ( 'NONE',  ( -91.89715655859116339, -275.8299030658744186, -321.9012202697894622 ) ) ;
#59625=CARTESIAN_POINT ( 'NONE',  ( 25.18347967487245143, -286.5347114446096839, -314.0067314835784487 ) ) ;
#59627=CARTESIAN_POINT ( 'NONE',  ( 4.054003918293396680, -288.6095584404092165, -207.7581160926768007 ) ) ;
#59628=CARTESIAN_POINT ( 'NONE',  ( -94.09131169823331220, -287.8695570592416857, -319.6511779892436493 ) ) ;
#59629=CARTESIAN_POINT ( 'NONE',  ( 33.55430200745949776, -282.7356276003422977, -288.7731642554599603 ) ) ;
#59630=CARTESIAN_POINT ( 'NONE',  ( -108.6987472884038226, -292.8588280642905488, -246.5718007206116908 ) ) ;
#59634=CARTESIAN_POINT ( 'NONE',  ( -35.88784722562734686, -299.9903649714495941, -194.8006387530634811 ) ) ;
#59635=CARTESIAN_POINT ( 'NONE',  ( 26.60492476982885179, -280.2644164302735703, -234.8163449392670827 ) ) ;
#59636=CARTESIAN_POINT ( 'NONE',  ( 20.88917038270630400, -280.2031966276928188, -317.6483226317695880 ) ) ;
#59637=CARTESIAN_POINT ( 'NONE',  ( -11.12194061459957339, -293.9162530564656208, -342.6441745598965554 ) ) ;
#59638=CARTESIAN_POINT ( 'NONE',  ( -110.1220644218794860, -270.9706115274059925, -256.6340620640322641 ) ) ;
#59639=CARTESIAN_POINT ( 'NONE',  ( 30.45590196705300912, -274.0382778421782746, -301.0987064551663934 ) ) ;
#59640=CARTESIAN_POINT ( 'NONE',  ( -69.92776676529885549, -296.8058422195309731, -336.2351776774651739 ) ) ;
#59642=CARTESIAN_POINT ( 'NONE',  ( -92.73242993315990645, -271.8519894405659443, -217.7067427971994675 ) ) ;
#59643=AXIS2_PLACEMENT_3D ( 'NONE', #49149, #78045, #65718 ) ;
#59644=CARTESIAN_POINT ( 'NONE',  ( -106.2568930367351214, -294.3768824206371164, -302.3715881081471366 ) ) ;
#59646=CARTESIAN_POINT ( 'NONE',  ( -17.28933198909028590, -293.7412133368897571, -199.5036038015535382 ) ) ;
#59648=CARTESIAN_POINT ( 'NONE',  ( 25.93744072116606958, -294.8576357937615740, -307.0810316534348772 ) ) ;
#59649=CARTESIAN_POINT ( 'NONE',  ( 129.4467878515196162, -293.3047352414760667, -195.3611179825600175 ) ) ;
#59650=CARTESIAN_POINT ( 'NONE',  ( -59.99100360468393944, -283.7803175849629156, -198.4359083877053820 ) ) ;
#59651=CARTESIAN_POINT ( 'NONE',  ( -108.4770382652945813, -296.7684173857288670, -253.9671048038309493 ) ) ;
#59653=CARTESIAN_POINT ( 'NONE',  ( -113.9038621022054798, -284.4496033952801213, -278.5608346757138065 ) ) ;
#59654=CARTESIAN_POINT ( 'NONE',  ( 21.73387225690156299, -282.8292874130477230, -223.2301447196631443 ) ) ;
#59655=CARTESIAN_POINT ( 'NONE',  ( -71.05314149151706715, -285.2860771790552121, -201.1564720917731961 ) ) ;
#59656=CARTESIAN_POINT ( 'NONE',  ( -105.7333461215181245, -288.1516246447949356, -300.8637023402644104 ) ) ;
#59657=CARTESIAN_POINT ( 'NONE',  ( -110.4542110544635705, -270.2666405000204009, -253.6410175316879361 ) ) ;
#59659=CARTESIAN_POINT ( 'NONE',  ( -5.570392078676166925, -285.1637882725778468, -204.0763753144603925 ) ) ;
#59660=CARTESIAN_POINT ( 'NONE',  ( -113.5082482855353305, -289.3545551430068485, -279.7527184563340370 ) ) ;
#59662=CARTESIAN_POINT ( 'NONE',  ( -68.84047990809658302, -297.0733918637204169, -337.1152956874589108 ) ) ;
#59663=CARTESIAN_POINT ( 'NONE',  ( -94.53291741035803852, -280.6692177007316218, -219.6879400736447394 ) ) ;
#59664=CARTESIAN_POINT ( 'NONE',  ( 24.35321449964746421, -292.1571913053898584, -313.6519101550778714 ) ) ;
#59665=CARTESIAN_POINT ( 'NONE',  ( 26.47937723959200085, -280.7338922373175478, -234.8793258868038265 ) ) ;
#59666=CARTESIAN_POINT ( 'NONE',  ( -58.84928545343898065, -295.4894442195571287, -344.3519570706346826 ) ) ;
#59667=CARTESIAN_POINT ( 'NONE',  ( -82.39725204952947024, -283.5227092671875084, -209.6385595715272814 ) ) ;
#59668=CARTESIAN_POINT ( 'NONE',  ( -56.08218604468325452, -281.8110800861148846, -197.6866429753504804 ) ) ;
#59669=CARTESIAN_POINT ( 'NONE',  ( -20.80666647776518019, -293.8935415776381319, -341.7576321749751855 ) ) ;
#59670=CARTESIAN_POINT ( 'NONE',  ( -15.51135221623666283, -296.3252638725264774, -195.3685521545008896 ) ) ;
#59673=CARTESIAN_POINT ( 'NONE',  ( 31.52959223255893306, -283.1544049475468796, -241.5758459045207758 ) ) ;
#59674=CARTESIAN_POINT ( 'NONE',  ( -70.96469589637160880, -295.0159718692639785, -335.2402254005137934 ) ) ;
#59676=CARTESIAN_POINT ( 'NONE',  ( -85.33152481854864391, -275.1952119285918457, -330.4860931364850671 ) ) ;
#59677=CARTESIAN_POINT ( 'NONE',  ( 24.35633267017240300, -274.1391117541636504, -224.5625200809061823 ) ) ;
#59678=CARTESIAN_POINT ( 'NONE',  ( 39.14665404777217361, -288.8461503707620182, -268.6788733772784781 ) ) ;
#59679=CARTESIAN_POINT ( 'NONE',  ( -108.9391484479606049, -290.1967658601028575, -284.6660408647016993 ) ) ;
#59680=CARTESIAN_POINT ( 'NONE',  ( -34.30394467215880638, -281.6111237512004095, -196.7177564679887212 ) ) ;
#59681=CARTESIAN_POINT ( 'NONE',  ( -87.89599776518949170, -274.9316707205931607, -216.5258683746128554 ) ) ;
#59682=CARTESIAN_POINT ( 'NONE',  ( -95.91943023011107528, -277.9652002268731508, -226.1160595509714994 ) ) ;
#59683=CARTESIAN_POINT ( 'NONE',  ( -54.38430306434025852, -279.2711085200696175, -343.4526894459543200 ) ) ;
#59685=CARTESIAN_POINT ( 'NONE',  ( -29.83677167309599199, -273.9779991765897762, -193.7277306544036435 ) ) ;
#59686=CARTESIAN_POINT ( 'NONE',  ( -67.16296899571523227, -293.5782509571520222, -202.1555014740926026 ) ) ;
#59690=CARTESIAN_POINT ( 'NONE',  ( 5.812442842206622551, -290.7699256440089357, -208.0873239530056651 ) ) ;
#59691=CARTESIAN_POINT ( 'NONE',  ( -103.2579016783744379, -272.4856301571839481, -238.8485361360083914 ) ) ;
#59692=DIRECTION ( 'NONE',  ( -1.000000000000000000, -0.000000000000000000, -0.000000000000000000 ) ) ;
#59693=CARTESIAN_POINT ( 'NONE',  ( 3.751701049364114748, -294.1141798777090912, -206.0019945936297461 ) ) ;
#59694=CARTESIAN_POINT ( 'NONE',  ( 35.59421657381088266, -301.4082689599840705, -190.3320873922940848 ) ) ;
#59695=CARTESIAN_POINT ( 'NONE',  ( -22.11098025402440470, -288.2477330025578794, -197.0409362066403389 ) ) ;
#59696=CARTESIAN_POINT ( 'NONE',  ( -35.08729803370692935, -275.0236121238818328, -345.1604903106862707 ) ) ;
#59697=CARTESIAN_POINT ( 'NONE',  ( 37.08210012868024563, -277.4522209368880112, -268.8080081081959065 ) ) ;
#59698=CARTESIAN_POINT ( 'NONE',  ( -63.28002308655479879, -289.7914272431645486, -200.5863546384857727 ) ) ;
#59699=CARTESIAN_POINT ( 'NONE',  ( -61.67373556538015578, -281.5998601866348849, -198.5544220683409264 ) ) ;
#59701=CARTESIAN_POINT ( 'NONE',  ( -45.65929330511178108, -282.5087999961667151, -343.0393846683190304 ) ) ;
#59702=CARTESIAN_POINT ( 'NONE',  ( -62.29237663306363260, -278.4487675711058614, -342.9358578157461466 ) ) ;
#59703=CARTESIAN_POINT ( 'NONE',  ( -34.50909818345874669, -281.8122183338728064, -346.9116574040626233 ) ) ;
#59705=CARTESIAN_POINT ( 'NONE',  ( -31.45630831760752599, -277.9209374053632473, -346.9523442054671136 ) ) ;
#59707=CARTESIAN_POINT ( 'NONE',  ( 20.30925315795902364, -277.7540913384030432, -320.3716528631812821 ) ) ;
#59708=CARTESIAN_POINT ( 'NONE',  ( -82.13390479932378696, -281.9090924074130839, -214.2458315076590907 ) ) ;
#59710=CARTESIAN_POINT ( 'NONE',  ( -111.2509992310975235, -298.7159470469808866, -257.6168582356684169 ) ) ;
#59711=CARTESIAN_POINT ( 'NONE',  ( -18.38034989409230846, -289.8818603630846837, -341.2284281143449789 ) ) ;
#59712=CARTESIAN_POINT ( 'NONE',  ( -37.84561078348364305, -275.0785680327639966, -345.0169544141380129 ) ) ;
#59713=CARTESIAN_POINT ( 'NONE',  ( -29.06498055141730674, -290.7089034677928794, -345.9485017376171641 ) ) ;
#59714=CARTESIAN_POINT ( 'NONE',  ( -2.383402299832444449, -291.8762109097629605, -206.1455775915851802 ) ) ;
#59715=CARTESIAN_POINT ( 'NONE',  ( 24.08928756656527881, -287.6771396316802907, -316.6834738628915034 ) ) ;
#59717=CARTESIAN_POINT ( 'NONE',  ( -89.47368205301026478, -282.2011493925952550, -322.6697982116314165 ) ) ;
#59718=CARTESIAN_POINT ( 'NONE',  ( -109.5464092174098596, -292.1888584972708713, -287.6048260822874454 ) ) ;
#59719=CARTESIAN_POINT ( 'NONE',  ( -106.2060208455930876, -283.3790556268481282, -244.1234907382296058 ) ) ;
#59720=CARTESIAN_POINT ( 'NONE',  ( 17.41916186665769573, -282.1707439834014508, -221.3459012405685655 ) ) ;
#59721=CARTESIAN_POINT ( 'NONE',  ( 14.45381702192093343, -289.2862508021310646, -327.0904162859282565 ) ) ;
#59722=CARTESIAN_POINT ( 'NONE',  ( -110.3413688935416701, -279.0048800858978097, -273.3672453267885203 ) ) ;
#59723=CARTESIAN_POINT ( 'NONE',  ( 21.01795744746100780, -291.6744495375634187, -220.7209254567658263 ) ) ;
#59725=CARTESIAN_POINT ( 'NONE',  ( -26.65370208993070733, -286.9875079116935694, -194.2161716983249278 ) ) ;
#59726=CARTESIAN_POINT ( 'NONE',  ( 25.80479491593573371, -288.6268492442459319, -314.4076601279724628 ) ) ;
#59727=CARTESIAN_POINT ( 'NONE',  ( -64.05339574406613679, -283.5772309151163881, -338.2984812065489564 ) ) ;
#59730=CARTESIAN_POINT ( 'NONE',  ( -55.90938056640048615, -293.6761043470941672, -196.8526613169327391 ) ) ;
#59731=CARTESIAN_POINT ( 'NONE',  ( 37.58421457211225913, -292.4317391272521718, -285.8338546751198237 ) ) ;
#59732=CARTESIAN_POINT ( 'NONE',  ( -68.14727241555689830, -276.5256521572768520, -336.8160517478360134 ) ) ;
#59733=CARTESIAN_POINT ( 'NONE',  ( -34.75535411046524104, -297.4323273630881204, -193.4633272928202246 ) ) ;
#59734=CARTESIAN_POINT ( 'NONE',  ( 9.302512522018274055, -291.1860493713606957, -213.2420877315347809 ) ) ;
#59735=CARTESIAN_POINT ( 'NONE',  ( -86.76047310469942886, -295.5934035755619789, -215.2633967151891454 ) ) ;
#59736=CARTESIAN_POINT ( 'NONE',  ( -36.21534744610778489, -293.2716266669405059, -196.9601422330328262 ) ) ;
#59737=CARTESIAN_POINT ( 'NONE',  ( 33.74917465839161679, -294.8670318935711521, -288.2584249475976321 ) ) ;
#59739=CARTESIAN_POINT ( 'NONE',  ( 30.56262401808909601, -291.9765684392257299, -302.7163727456934339 ) ) ;
#59740=CARTESIAN_POINT ( 'NONE',  ( -90.66203747850281047, -299.2970177042143973, -217.5448304489311226 ) ) ;
#59741=CARTESIAN_POINT ( 'NONE',  ( 33.61355940060740721, -288.2542460067980414, -252.1788055280051992 ) ) ;
#59742=CARTESIAN_POINT ( 'NONE',  ( 26.27410627145429345, -278.0740542999984086, -310.8492002204433788 ) ) ;
#59743=CARTESIAN_POINT ( 'NONE',  ( -48.03319200387923615, -278.6038275693235846, -194.5514960662683279 ) ) ;
#59745=CARTESIAN_POINT ( 'NONE',  ( -58.08613152476248587, -273.1396816699996180, -196.2586118664796686 ) ) ;
#59746=CARTESIAN_POINT ( 'NONE',  ( 22.14621409499660487, -280.2484827093200579, -315.1315004234939465 ) ) ;
#59747=CARTESIAN_POINT ( 'NONE',  ( -56.33732028574098649, -278.2113705855249464, -196.5123383668334611 ) ) ;
#59748=EDGE_CURVE ( 'NONE', #33611, #82501, #4861, .T. ) ;
#59749=CARTESIAN_POINT ( 'NONE',  ( -105.4250072226659256, -294.8687517528945818, -298.0361387046005461 ) ) ;
#59751=CARTESIAN_POINT ( 'NONE',  ( 21.55839628155816001, -275.5977646934261998, -227.0636433290985678 ) ) ;
#59753=CARTESIAN_POINT ( 'NONE',  ( -110.3936965504984897, -288.8092463544043653, -251.8210390098774667 ) ) ;
#59754=CARTESIAN_POINT ( 'NONE',  ( -87.38443519962841322, -289.7274506397511118, -328.9522982916945466 ) ) ;
#59755=CARTESIAN_POINT ( 'NONE',  ( -35.59260432212233383, -276.0741778146834235, -195.2019822268128451 ) ) ;
#59756=CARTESIAN_POINT ( 'NONE',  ( -111.0780818667128642, -294.7162722516676467, -257.5949738405867038 ) ) ;
#59757=CARTESIAN_POINT ( 'NONE',  ( 2.002657579084959671, -281.7366859000046020, -336.3624841579058398 ) ) ;
#59758=DIRECTION ( 'NONE',  ( 0.000000000000000000, 0.000000000000000000, -1.000000000000000000 ) ) ;
#59759=CARTESIAN_POINT ( 'NONE',  ( 34.57257919619672037, -279.8267546078670875, -291.6975797765239804 ) ) ;
#59761=CARTESIAN_POINT ( 'NONE',  ( -105.4873961128336219, -288.9825365149166601, -297.7610262616169621 ) ) ;
#59762=CARTESIAN_POINT ( 'NONE',  ( -72.00631184373531823, -281.6552263192173200, -336.0058449377789316 ) ) ;
#59765=CARTESIAN_POINT ( 'NONE',  ( 10.13402971821695076, -290.7060881081154662, -212.2329443478662370 ) ) ;
#59766=CARTESIAN_POINT ( 'NONE',  ( -73.21322283195371483, -279.1362628165799151, -334.8711922747243648 ) ) ;
#59767=CARTESIAN_POINT ( 'NONE',  ( -78.93120839027876912, -284.8046296929813366, -334.6909051766065772 ) ) ;
#59768=CARTESIAN_POINT ( 'NONE',  ( 24.97114220135220464, -273.0570098735959732, -227.6014939173690550 ) ) ;
#59769=CARTESIAN_POINT ( 'NONE',  ( -41.32292902932859135, -286.0006676799977186, -197.4572633832124495 ) ) ;
#59770=CARTESIAN_POINT ( 'NONE',  ( 10.05731441514111957, -277.8089130592833840, -326.6523991530547733 ) ) ;
#59771=CARTESIAN_POINT ( 'NONE',  ( 22.60400914789265769, -276.9396298768385236, -312.3898986367362909 ) ) ;
#59772=CARTESIAN_POINT ( 'NONE',  ( -110.4169716308812070, -286.7690747041713166, -253.4790165613358113 ) ) ;
#59775=CARTESIAN_POINT ( 'NONE',  ( -111.5925811222122945, -296.1300434154398431, -290.7524562445588003 ) ) ;
#59776=CARTESIAN_POINT ( 'NONE',  ( -7.622748016606969657, -288.4235515614760743, -201.8875413966727024 ) ) ;
#59778=CARTESIAN_POINT ( 'NONE',  ( 25.18497378105905682, -285.6952119285918457, -320.2651865833026363 ) ) ;
#59779=CARTESIAN_POINT ( 'NONE',  ( -90.83267612166100946, -278.2353242451486039, -215.3306785861155390 ) ) ;
#59780=CARTESIAN_POINT ( 'NONE',  ( -85.98650101412113145, -289.7912209694848116, -211.6400533138141782 ) ) ;
#59781=CARTESIAN_POINT ( 'NONE',  ( -110.1088070768855403, -286.2255244645986636, -258.6339156118998517 ) ) ;
#59783=CARTESIAN_POINT ( 'NONE',  ( -111.1775206948295249, -280.2365831447859250, -276.1805726540234787 ) ) ;
#59784=CARTESIAN_POINT ( 'NONE',  ( 38.20027581120578475, -288.8315202155641828, -258.7843080269046823 ) ) ;
#59785=CARTESIAN_POINT ( 'NONE',  ( -20.92632432880489191, -284.8417872597761971, -343.5960877921627912 ) ) ;
#59786=CARTESIAN_POINT ( 'NONE',  ( 3.503300492076803607, -276.6860664231760438, -335.6978129411951954 ) ) ;
#59787=CARTESIAN_POINT ( 'NONE',  ( -69.95388855377572668, -295.6405455579798627, -203.2173023830663965 ) ) ;
#59788=CARTESIAN_POINT ( 'NONE',  ( -79.90901449609418705, -279.3272215037501951, -206.1331212874697769 ) ) ;
#59789=CARTESIAN_POINT ( 'NONE',  ( -105.0381334677153546, -298.8832036626652098, -239.2771928253048657 ) ) ;
#59791=CARTESIAN_POINT ( 'NONE',  ( -69.91165696735023971, -276.1233781216988064, -202.8022627189028810 ) ) ;
#59792=CARTESIAN_POINT ( 'NONE',  ( -85.15302759674364097, -271.6420913858016206, -211.3013941687038084 ) ) ;
#59794=CARTESIAN_POINT ( 'NONE',  ( -48.62352373873373068, -276.7071936022409773, -342.5977910885592905 ) ) ;
#59795=CARTESIAN_POINT ( 'NONE',  ( -73.76964031996159576, -274.7849751319397456, -202.9151006532376016 ) ) ;
#59796=CARTESIAN_POINT ( 'NONE',  ( -8.139531221201190547, -281.7378022744816235, -341.4108144909678799 ) ) ;
#59797=CARTESIAN_POINT ( 'NONE',  ( 22.79798817802251065, -289.9070913852672788, -313.5026513959310250 ) ) ;
#59798=CARTESIAN_POINT ( 'NONE',  ( -97.69758570922418528, -298.7014313077266934, -223.6508929627860596 ) ) ;
#59799=CARTESIAN_POINT ( 'NONE',  ( -51.74110041214319011, -299.0770784330292713, -195.0696592759014436 ) ) ;
#59800=CARTESIAN_POINT ( 'NONE',  ( -58.18952085651297779, -293.7824356915734825, -198.4362126842878808 ) ) ;
#59801=CARTESIAN_POINT ( 'NONE',  ( 32.02462957728457837, -279.9187893120579815, -298.4385239749499306 ) ) ;
#59802=CARTESIAN_POINT ( 'NONE',  ( 27.70551190340293957, -282.9869646775324554, -234.1647866440740415 ) ) ;
#59803=CARTESIAN_POINT ( 'NONE',  ( -97.59444279829156699, -271.1767109208637407, -226.2133471507214040 ) ) ;
#59804=CARTESIAN_POINT ( 'NONE',  ( -94.71878262826569994, -285.4669500191061502, -320.5040219714072123 ) ) ;
#59805=CARTESIAN_POINT ( 'NONE',  ( 14.29138804546174057, -287.2255620141465897, -322.4019700025412476 ) ) ;
#59806=CARTESIAN_POINT ( 'NONE',  ( 66.25670972154831873, 47.06390698321332167, -318.7317394719314620 ) ) ;
#59808=CARTESIAN_POINT ( 'NONE',  ( 7.573381283506060768, -287.0277106130403695, -332.2425486772297063 ) ) ;
#59809=CARTESIAN_POINT ( 'NONE',  ( 19.52728127439686645, -287.8662783969826364, -316.1651182568014633 ) ) ;
#59810=ORIENTED_EDGE ( 'NONE', *, *, #75831, .T. ) ;
#59811=CARTESIAN_POINT ( 'NONE',  ( -101.1542674085729345, -285.0685943038000119, -312.9939953919073332 ) ) ;
#59812=CARTESIAN_POINT ( 'NONE',  ( -4.098849446580143940, -274.8363442099954455, -205.3316957875819355 ) ) ;
#59813=CARTESIAN_POINT ( 'NONE',  ( -105.7222414134044612, -289.9226437226115536, -235.5224008523209136 ) ) ;
#59814=CARTESIAN_POINT ( 'NONE',  ( 37.76776037595595170, -282.4108126385665400, -286.9107941091407952 ) ) ;
#59815=CARTESIAN_POINT ( 'NONE',  ( 38.92742961939502067, -283.1024758045021485, -272.7543581536374973 ) ) ;
#59816=CARTESIAN_POINT ( 'NONE',  ( -71.72548637421012074, -283.8273894029236999, -339.2341862678035795 ) ) ;
#59817=CARTESIAN_POINT ( 'NONE',  ( -85.48418169845588466, -279.3641122505070484, -215.4857913935897500 ) ) ;
#59818=CARTESIAN_POINT ( 'NONE',  ( -54.42813229853333468, -271.3380690714489560, -195.3538533559490702 ) ) ;
#59819=CARTESIAN_POINT ( 'NONE',  ( 168.5485566325764069, 232.3890912981213717, -192.7980796144592546 ) ) ;
#59821=CARTESIAN_POINT ( 'NONE',  ( 36.42875546167547185, -277.3896077738209556, -257.7174078676169984 ) ) ;
#59822=CARTESIAN_POINT ( 'NONE',  ( 167.0956850759771157, 232.7156327414166697, -192.3491569821647147 ) ) ;
#59823=CARTESIAN_POINT ( 'NONE',  ( -35.13557503043015373, -297.4290726340713036, -197.2594361228370872 ) ) ;
#59824=CARTESIAN_POINT ( 'NONE',  ( 23.06366043742156791, -292.4217407343726336, -222.6879977926365370 ) ) ;
#59825=CARTESIAN_POINT ( 'NONE',  ( 197.1939414079961068, 281.6276418469664122, -110.3312364695952255 ) ) ;
#59826=CARTESIAN_POINT ( 'NONE',  ( -110.5602435304467832, -271.5193695338213047, -247.9913494692551978 ) ) ;
#59827=CARTESIAN_POINT ( 'NONE',  ( -15.63559332744059560, -287.1665590860283714, -340.9502193199492126 ) ) ;
#59828=CARTESIAN_POINT ( 'NONE',  ( -20.54606043807000759, -296.6947587259135162, -342.7243565857409635 ) ) ;
#59829=CARTESIAN_POINT ( 'NONE',  ( -62.74897468898124941, -287.0297092932822238, -201.3451565021675549 ) ) ;
#59831=CARTESIAN_POINT ( 'NONE',  ( -32.01682861958862247, -295.9277974261654549, -346.9541332634416904 ) ) ;
#59832=CARTESIAN_POINT ( 'NONE',  ( -103.5438792155005814, -285.4629318991974287, -239.3338853962637529 ) ) ;
#59833=CARTESIAN_POINT ( 'NONE',  ( 53.02061087099094294, -297.9547193582686191, -193.7761767739849859 ) ) ;
#59834=CARTESIAN_POINT ( 'NONE',  ( -44.89137728774763758, -292.7618475729618126, -193.8415738790481555 ) ) ;
#59835=CARTESIAN_POINT ( 'NONE',  ( 35.43025780430517813, -294.3613555150514003, -295.4997882179580984 ) ) ;
#59836=CARTESIAN_POINT ( 'NONE',  ( -69.01952119185894219, -291.7903132264139003, -204.5786621262338940 ) ) ;
#59839=CARTESIAN_POINT ( 'NONE',  ( -112.4343469585250119, -274.5792469029044582, -261.9701353890976634 ) ) ;
#59840=CARTESIAN_POINT ( 'NONE',  ( 11.54415370207408564, -273.5076165051057160, -211.3160649113189038 ) ) ;
#59843=CARTESIAN_POINT ( 'NONE',  ( 23.46555241426075611, -275.6899676316126033, -317.5206302212818059 ) ) ;
#59844=CARTESIAN_POINT ( 'NONE',  ( -98.49479361424627655, -271.5211272808954277, -228.9572805244135623 ) ) ;
#59845=CARTESIAN_POINT ( 'NONE',  ( -94.04883340816303416, -281.0822238220499116, -222.4336601087031511 ) ) ;
#59846=CARTESIAN_POINT ( 'NONE',  ( -4.541289912399062878, -274.7549574148200122, -336.9710266119130324 ) ) ;
#59847=CARTESIAN_POINT ( 'NONE',  ( -106.1835776299343905, -298.0965403650738494, -244.7600371908943657 ) ) ;
#59848=CARTESIAN_POINT ( 'NONE',  ( -78.99872674225353819, -274.4166242656008308, -210.0657947924567281 ) ) ;
#59849=CARTESIAN_POINT ( 'NONE',  ( -92.45286756839716702, -275.0368891145354837, -218.0283277660527119 ) ) ;
#59850=CARTESIAN_POINT ( 'NONE',  ( -60.34452159860159526, -271.7755938740722854, -198.5482201839979552 ) ) ;
#59851=CARTESIAN_POINT ( 'NONE',  ( 17.16209751502314518, -294.8996385466196557, -319.0957885185661667 ) ) ;
#59852=CARTESIAN_POINT ( 'NONE',  ( -69.25685667554330394, -290.1986187309854586, -204.0388515191822592 ) ) ;
#59853=CYLINDRICAL_SURFACE ( 'NONE', #35205, 1.895975569037589015 ) ;
#59854=CARTESIAN_POINT ( 'NONE',  ( -14.60189432618421179, -277.2575962254414321, -343.9181122100008565 ) ) ;
#59855=CARTESIAN_POINT ( 'NONE',  ( -35.39245437488732904, -274.2439415676043950, -197.3746416265469463 ) ) ;
#59857=CARTESIAN_POINT ( 'NONE',  ( -106.5665948135525980, -282.8170347997694876, -302.9373704866046069 ) ) ;
#59858=CARTESIAN_POINT ( 'NONE',  ( -30.72631281538588510, -296.9688542096346282, -345.2361143240630099 ) ) ;
#59860=CARTESIAN_POINT ( 'NONE',  ( 9.140943131670363542, -285.9068609658804689, -213.8636348349867262 ) ) ;
#59861=CARTESIAN_POINT ( 'NONE',  ( -30.40993362373118103, -280.9644985858088262, -345.2074875628674135 ) ) ;
#59862=CARTESIAN_POINT ( 'NONE',  ( -43.31085443167592786, -275.3684220568890737, -344.1333567353430567 ) ) ;
#59863=CARTESIAN_POINT ( 'NONE',  ( 30.81697159432768274, -274.4971626236555835, -298.2413610292055637 ) ) ;
#59864=CARTESIAN_POINT ( 'NONE',  ( 36.02782401972909554, -283.3518243804489316, -254.7468375708408814 ) ) ;
#59865=CARTESIAN_POINT ( 'NONE',  ( 24.11765056412005848, -276.2042337513098573, -230.2378240344406493 ) ) ;
#59868=CARTESIAN_POINT ( 'NONE',  ( -18.72548618634065321, -272.6877316019501336, -196.4156757316058020 ) ) ;
#59869=CARTESIAN_POINT ( 'NONE',  ( -31.24839846841152280, -282.1289783530559134, -195.3903910776010662 ) ) ;
#59871=CARTESIAN_POINT ( 'NONE',  ( -2.901492816105845751, -288.4237949380349164, -203.0920053168421475 ) ) ;
#59873=CARTESIAN_POINT ( 'NONE',  ( -62.51885965831366576, -287.3794356077967791, -341.0632713737886093 ) ) ;
#59874=CARTESIAN_POINT ( 'NONE',  ( 82.12341071034305173, -301.5530703083973094, -195.5810619036753621 ) ) ;
#59875=CARTESIAN_POINT ( 'NONE',  ( -110.8342274447078353, -271.2731220238221681, -267.6021512995649800 ) ) ;
#59876=CARTESIAN_POINT ( 'NONE',  ( -96.07740985483196994, -289.3203087400980280, -224.9630796293529613 ) ) ;
#59877=CARTESIAN_POINT ( 'NONE',  ( -112.8394912670188432, -266.8193566212495966, -283.2716462811306428 ) ) ;
#59879=CARTESIAN_POINT ( 'NONE',  ( 23.57690612498094040, -286.6495310681497131, -316.3136061280771401 ) ) ;
#59880=CARTESIAN_POINT ( 'NONE',  ( -4.452535808313517585, -284.2113900780484528, -336.4273218072285090 ) ) ;
#59881=CARTESIAN_POINT ( 'NONE',  ( -107.3030483509968604, -282.4079987788808808, -300.1502239984573066 ) ) ;
#59882=CARTESIAN_POINT ( 'NONE',  ( -70.22071680094495605, -291.6062597767686952, -205.1846631646922390 ) ) ;
#59883=CARTESIAN_POINT ( 'NONE',  ( 20.65648588179590917, -283.6107212219213238, -315.6555474253764260 ) ) ;
#59884=CARTESIAN_POINT ( 'NONE',  ( -7.177580718275951455, -283.4488846991008018, -337.0286522395519455 ) ) ;
#59885=CARTESIAN_POINT ( 'NONE',  ( -54.11052887803349165, -291.2461902545247199, -343.8803853110682667 ) ) ;
#59886=CARTESIAN_POINT ( 'NONE',  ( -96.92240829427498738, -273.5402224874503077, -221.5975117940554640 ) ) ;
#59887=CARTESIAN_POINT ( 'NONE',  ( -3.723798878786034994, -286.6919988280857865, -338.0448949012799744 ) ) ;
#59888=CARTESIAN_POINT ( 'NONE',  ( 36.06263233575805316, -275.8444448026766622, -293.6163104250691163 ) ) ;
#59889=CARTESIAN_POINT ( 'NONE',  ( -87.04257176165499743, -293.3364210459879473, -214.5988856252446340 ) ) ;
#59891=CARTESIAN_POINT ( 'NONE',  ( 35.77081079830085031, -277.8376638359845288, -253.6410175316879361 ) ) ;
#59892=CARTESIAN_POINT ( 'NONE',  ( -48.25363108850776683, -275.1904010751892429, -344.7841434390111317 ) ) ;
#59894=CARTESIAN_POINT ( 'NONE',  ( -98.43866940082922667, -295.5643255791685533, -224.8025413472602168 ) ) ;
#59895=CARTESIAN_POINT ( 'NONE',  ( -55.22572924904498137, -293.4183893965025050, -198.7608252775363837 ) ) ;
#59896=CARTESIAN_POINT ( 'NONE',  ( -85.37089824739111066, -272.7164044348450034, -215.1838689634349748 ) ) ;
#59897=CARTESIAN_POINT ( 'NONE',  ( -111.0618844352059540, -292.0970852283807631, -268.4630347558305061 ) ) ;
#59898=CARTESIAN_POINT ( 'NONE',  ( -22.70528133408100757, -293.1853659735446058, -198.6033052213029180 ) ) ;
#59899=CARTESIAN_POINT ( 'NONE',  ( -101.8858418863424617, -286.8023473990782577, -234.0341057589306502 ) ) ;
#59900=CARTESIAN_POINT ( 'NONE',  ( 27.54234683659478478, -294.4442714519171886, -229.9044345564421121 ) ) ;
#59901=CARTESIAN_POINT ( 'NONE',  ( 24.49762168190883571, -295.4692711078989191, -315.4297960445541094 ) ) ;
#59902=CARTESIAN_POINT ( 'NONE',  ( -13.01024369078865384, -294.5604493792727112, -339.2400989432494498 ) ) ;
#59903=CARTESIAN_POINT ( 'NONE',  ( 14.50420669101167093, -288.7812082875682904, -216.0953726551335023 ) ) ;
#59904=CARTESIAN_POINT ( 'NONE',  ( 0.8702025466675872289, -282.7237271127066833, -337.2258118303606125 ) ) ;
#59905=CARTESIAN_POINT ( 'NONE',  ( 73.76994744378262681, -297.5125299601920119, -194.8371112144576216 ) ) ;
#59906=CARTESIAN_POINT ( 'NONE',  ( -46.50339244953634221, -285.7722435388460553, -193.9081036645936820 ) ) ;
#59907=CARTESIAN_POINT ( 'NONE',  ( 26.80156856705642809, -278.0453233320057507, -308.5381776122274573 ) ) ;
#59908=CARTESIAN_POINT ( 'NONE',  ( -96.88802799567245927, -283.9441705592350900, -227.4285498773733707 ) ) ;
#59909=CARTESIAN_POINT ( 'NONE',  ( 35.77570596229903543, -285.3369260600396728, -253.6053634102506464 ) ) ;
#59910=CARTESIAN_POINT ( 'NONE',  ( -28.34773591233913592, -278.3045522671701519, -195.0792745551300129 ) ) ;
#59912=CARTESIAN_POINT ( 'NONE',  ( -66.58996174927615641, -282.9535259265710465, -337.3263824336396510 ) ) ;
#59913=CARTESIAN_POINT ( 'NONE',  ( -77.29856545092492581, -280.7343952382271368, -204.9433145908795950 ) ) ;
#59914=CARTESIAN_POINT ( 'NONE',  ( 29.93115793733951335, -286.1293350021964557, -233.2753574517882100 ) ) ;
#59915=CARTESIAN_POINT ( 'NONE',  ( 25.29665154043909325, -295.8505621639567380, -309.8834532017362449 ) ) ;
#59916=CARTESIAN_POINT ( 'NONE',  ( -77.37706367951381026, -279.1793560791526261, -335.2576795012071784 ) ) ;
#59918=CARTESIAN_POINT ( 'NONE',  ( -12.01354245582624714, -278.0445835991639001, -342.6093692790500427 ) ) ;
#59919=CARTESIAN_POINT ( 'NONE',  ( -109.2864456931788055, -278.2213494960535058, -282.8024568442604618 ) ) ;
#59921=CARTESIAN_POINT ( 'NONE',  ( -95.90150665561472465, -299.1941044623279709, -223.7695147596665493 ) ) ;
#59922=CARTESIAN_POINT ( 'NONE',  ( 37.38498537389749288, -285.4893312287964022, -265.4921790455068162 ) ) ;
#59924=CARTESIAN_POINT ( 'NONE',  ( -99.20870705545418389, -291.5561715330583183, -314.8684501775746867 ) ) ;
#59925=CARTESIAN_POINT ( 'NONE',  ( -47.85088403527714007, -294.1091254032806432, -342.9645502403151340 ) ) ;
#59927=CARTESIAN_POINT ( 'NONE',  ( 14.32824189675854853, -293.9681046555747344, -322.0297335270641952 ) ) ;
#59929=CARTESIAN_POINT ( 'NONE',  ( -113.8802116867503145, -291.6924967883056752, -265.5290627889569350 ) ) ;
#59930=CARTESIAN_POINT ( 'NONE',  ( -41.06466110886249510, -280.6554759195682891, -197.3540482569941048 ) ) ;
#59931=CARTESIAN_POINT ( 'NONE',  ( -70.02067741567400105, -272.6909438608519736, -200.8852158456117820 ) ) ;
#59932=CARTESIAN_POINT ( 'NONE',  ( 36.59091332883427583, -287.9359521538286799, -249.0230873958698794 ) ) ;
#59933=CARTESIAN_POINT ( 'NONE',  ( 27.42930485019983067, -288.4324054879674577, -312.0582237548915714 ) ) ;
#59934=CARTESIAN_POINT ( 'NONE',  ( -110.2496245091570728, -284.9499649275306297, -265.4680148169834411 ) ) ;
#59936=CARTESIAN_POINT ( 'NONE',  ( -100.6316193246363895, -246.5931397093643795, -333.0237302267296400 ) ) ;
#59937=CARTESIAN_POINT ( 'NONE',  ( -39.45748113467511331, -139.8532795829076463, -360.8829801073189856 ) ) ;
#59938=CARTESIAN_POINT ( 'NONE',  ( -8.684830022753116552, -275.8644938294555118, -337.6902561242339402 ) ) ;
#59939=CARTESIAN_POINT ( 'NONE',  ( -93.85306733370345000, -276.8130911310531701, -317.0786652712330920 ) ) ;
#59940=CARTESIAN_POINT ( 'NONE',  ( -34.75570499637699129, -297.5913720358046248, -193.4228652938332687 ) ) ;
#59941=CARTESIAN_POINT ( 'NONE',  ( -104.5598740624659513, -261.7493365748397878, -316.1504158153062463 ) ) ;
#59942=CARTESIAN_POINT ( 'NONE',  ( -98.15842529236812197, -290.4826491639692563, -310.8723386717459789 ) ) ;
#59943=CARTESIAN_POINT ( 'NONE',  ( 19.23069837402722371, -299.5463773817224364, -193.5150897415832105 ) ) ;
#59944=CARTESIAN_POINT ( 'NONE',  ( -95.01552854323075792, -273.8931649452441093, -219.4981422270397502 ) ) ;
#59945=CARTESIAN_POINT ( 'NONE',  ( -107.8362130380808281, -296.9698491233963296, -251.3518349678664947 ) ) ;
#59946=ORIENTED_EDGE ( 'NONE', *, *, #65700, .T. ) ;
#59948=CARTESIAN_POINT ( 'NONE',  ( -102.3541008922031921, -279.9599116326868966, -308.9695364781742342 ) ) ;
#59949=CARTESIAN_POINT ( 'NONE',  ( -31.64710392622223267, -282.4897672494021208, -347.1018050768863077 ) ) ;
#59951=CARTESIAN_POINT ( 'NONE',  ( -91.18557997915989688, -278.9196045203940457, -320.1849426367939486 ) ) ;
#59952=CARTESIAN_POINT ( 'NONE',  ( -98.81658237866699324, -279.7115242311438124, -315.0465626485628263 ) ) ;
#59953=CARTESIAN_POINT ( 'NONE',  ( -70.71870656527912047, -296.1777577622423223, -204.7624146363433226 ) ) ;
#59956=CARTESIAN_POINT ( 'NONE',  ( -9.249308301015997102, -280.5966293190467695, -202.9829499609261063 ) ) ;
#59957=CARTESIAN_POINT ( 'NONE',  ( 19.76405880992443187, -277.0544565268701831, -321.7918136389699839 ) ) ;
#59958=CARTESIAN_POINT ( 'NONE',  ( 28.18736872967216556, -277.0655372054245049, -233.7723145199266241 ) ) ;
#59959=CARTESIAN_POINT ( 'NONE',  ( -3.006269638561347879, -275.1822099983924659, -338.6375640229837245 ) ) ;
#59962=CARTESIAN_POINT ( 'NONE',  ( -25.37262622998626327, -291.4056441699275410, -198.1337458989947606 ) ) ;
#59963=CARTESIAN_POINT ( 'NONE',  ( 16.23412307829809365, -286.1374419462657102, -215.1982323242311566 ) ) ;
#59964=CARTESIAN_POINT ( 'NONE',  ( -37.56579216964176027, -281.2948887900610089, -344.3867177952171232 ) ) ;
#59965=CARTESIAN_POINT ( 'NONE',  ( -56.48956269030360033, -281.8785408671863593, -341.4155638312459473 ) ) ;
#59966=CARTESIAN_POINT ( 'NONE',  ( 20.65215831188271878, -284.9847601820686691, -223.6715820239177503 ) ) ;
#59967=CARTESIAN_POINT ( 'NONE',  ( 23.65080172314155149, -290.1469955183363254, -314.0927358630821686 ) ) ;
#59968=CARTESIAN_POINT ( 'NONE',  ( 19.97653418451871232, -282.1130215345847319, -224.5162652557175136 ) ) ;
#59969=CARTESIAN_POINT ( 'NONE',  ( -102.4795565685557790, -271.0489455320371803, -233.0808819269815046 ) ) ;
#59970=CARTESIAN_POINT ( 'NONE',  ( -3.269032450612306739, -281.0096783425094031, -338.5334763367176834 ) ) ;
#59971=CARTESIAN_POINT ( 'NONE',  ( 9.957276081149519342, -296.4011405635624783, -328.6329376264565099 ) ) ;
#59972=CARTESIAN_POINT ( 'NONE',  ( -40.93771608963155018, -278.2473815861245043, -194.4465631866245587 ) ) ;
#59973=CARTESIAN_POINT ( 'NONE',  ( -108.8627853391299709, -279.0043819126972267, -285.4815359254573650 ) ) ;
#59974=CARTESIAN_POINT ( 'NONE',  ( -112.4947376363317915, -286.5925953426739738, -267.2171151802833720 ) ) ;
#59976=CARTESIAN_POINT ( 'NONE',  ( -91.79169301609626075, -293.2037747349238543, -217.8985594117043547 ) ) ;
#59977=CARTESIAN_POINT ( 'NONE',  ( -6.713583523252705021, -274.6499094297258239, -338.8221954292720284 ) ) ;
#59978=CARTESIAN_POINT ( 'NONE',  ( 33.88878854897261306, -287.1175407733646807, -299.3190446538386595 ) ) ;
#59979=CARTESIAN_POINT ( 'NONE',  ( -3.248766159620207539, -290.9101817495467799, -204.9079876501931494 ) ) ;
#59980=DIRECTION ( 'NONE',  ( 0.000000000000000000, 0.000000000000000000, -1.000000000000000000 ) ) ;
#59981=CARTESIAN_POINT ( 'NONE',  ( -54.08243044369199026, -275.9563074602513666, -341.9747163648090691 ) ) ;
#59982=CARTESIAN_POINT ( 'NONE',  ( -96.60448239626387590, -294.0739507885874104, -315.0898748861079071 ) ) ;
#59983=CARTESIAN_POINT ( 'NONE',  ( -108.9115299702456667, -292.0869143084013899, -253.6028031454002871 ) ) ;
#59985=CARTESIAN_POINT ( 'NONE',  ( -7.443854635798750508, -290.9169794872181001, -200.1413211783660131 ) ) ;
#59986=CARTESIAN_POINT ( 'NONE',  ( 35.78604678410714968, -289.0177414312382780, -260.0501408862831454 ) ) ;
#59987=CARTESIAN_POINT ( 'NONE',  ( -112.1701820300762762, -288.9595082875632670, -257.1447527013571062 ) ) ;
#59988=CARTESIAN_POINT ( 'NONE',  ( 7.269833936686640463, -288.0986812405787987, -211.7716587364999157 ) ) ;
#59990=CARTESIAN_POINT ( 'NONE',  ( 33.18220331233044362, -288.0983141563156664, -250.8936895230266089 ) ) ;
#59991=CARTESIAN_POINT ( 'NONE',  ( -1.466534964591752699, -296.5588674342830018, -336.6431706760815814 ) ) ;
#59992=CARTESIAN_POINT ( 'NONE',  ( 82.64890176555634582, -299.5541904835138780, -197.7570935515976203 ) ) ;
#59993=CARTESIAN_POINT ( 'NONE',  ( 36.76420277686428051, -289.0013069038577669, -289.7601868853059841 ) ) ;
#59994=CARTESIAN_POINT ( 'NONE',  ( -72.96533557734936437, -277.6026813209381316, -203.9434512651407658 ) ) ;
#59995=CARTESIAN_POINT ( 'NONE',  ( -38.54037258048894898, -277.4000767044311715, -347.3306410159770508 ) ) ;
#59996=CARTESIAN_POINT ( 'NONE',  ( -8.864986838942877867, -280.0813804991981328, -198.8431405798105800 ) ) ;
#59997=CARTESIAN_POINT ( 'NONE',  ( -44.75701922743524364, -299.9378694268813774, -196.0340335865562054 ) ) ;
#59998=CARTESIAN_POINT ( 'NONE',  ( -49.72740002051758523, -283.8941529133288668, -196.3379803099534229 ) ) ;
#60000=CARTESIAN_POINT ( 'NONE',  ( -34.23837009260996922, -278.2311321860943281, -196.1780528109326838 ) ) ;
#60001=CARTESIAN_POINT ( 'NONE',  ( -52.53794309811355134, -281.2465061557251715, -343.8585641416272551 ) ) ;
#60003=CARTESIAN_POINT ( 'NONE',  ( -77.46693802465658507, -276.0596087175227922, -335.3276371634951261 ) ) ;
#60004=CARTESIAN_POINT ( 'NONE',  ( -80.54575753980547859, -297.1701315814090663, -330.0613455692244429 ) ) ;
#60005=CARTESIAN_POINT ( 'NONE',  ( 37.24451121664420583, -280.6971994382673756, -288.2605650847006586 ) ) ;
#60006=CARTESIAN_POINT ( 'NONE',  ( -110.3326625622826782, -297.4069985505269642, -276.9326452309686033 ) ) ;
#60007=CARTESIAN_POINT ( 'NONE',  ( -112.9638697334090125, -274.1199723198372453, -259.0500456937389231 ) ) ;
#60008=CARTESIAN_POINT ( 'NONE',  ( -0.5319458963451971778, -274.2225929373191775, -207.2820357615500768 ) ) ;
#60009=CARTESIAN_POINT ( 'NONE',  ( 30.20663376833570979, -295.9829947566333317, -303.0727378157774297 ) ) ;
#60010=CARTESIAN_POINT ( 'NONE',  ( 9.809080576523538042, -286.8480423831206849, -209.4858037457485409 ) ) ;
#60011=CARTESIAN_POINT ( 'NONE',  ( -92.01459899129939402, -277.3594001382181773, -218.1309640287522882 ) ) ;
#60012=CARTESIAN_POINT ( 'NONE',  ( -89.49304150174650374, -289.5965242215511353, -327.0112512340981539 ) ) ;
#60014=CARTESIAN_POINT ( 'NONE',  ( -66.43349028916553323, -288.5013157416526042, -337.6245103654333661 ) ) ;
#60015=CARTESIAN_POINT ( 'NONE',  ( 22.39803500793282609, -290.9314232945565664, -224.9950232031948474 ) ) ;
#60018=CARTESIAN_POINT ( 'NONE',  ( -78.21402997820378289, -289.1256732226037798, -330.9814285970900301 ) ) ;
#60020=CARTESIAN_POINT ( 'NONE',  ( -49.31987434615352583, -286.8444318614805866, -194.4831196181479527 ) ) ;
#60021=CARTESIAN_POINT ( 'NONE',  ( 17.36665895637874613, -295.4090924074130839, -226.6919474004047572 ) ) ;
#60022=CARTESIAN_POINT ( 'NONE',  ( 31.97866207542431738, -292.1855170949002627, -237.2601640534593912 ) ) ;
#60023=EDGE_CURVE ( 'NONE', #46969, #57853, #55465, .T. ) ;
#60024=CARTESIAN_POINT ( 'NONE',  ( -58.33524340190015067, -284.6330159097171304, -343.9864239888361794 ) ) ;
#60025=CARTESIAN_POINT ( 'NONE',  ( -58.95015643619222345, -283.1728226824019430, -340.1428384657923516 ) ) ;
#60026=CARTESIAN_POINT ( 'NONE',  ( -91.63552747125348219, -297.3041668406910958, -215.7609319716147809 ) ) ;
#60027=CARTESIAN_POINT ( 'NONE',  ( 34.85483683740542915, -276.6872371516304838, -256.6168999520595548 ) ) ;
#60028=CARTESIAN_POINT ( 'NONE',  ( -36.15525363930201053, -290.0871741326099027, -195.7129860930606355 ) ) ;
#60029=CARTESIAN_POINT ( 'NONE',  ( 32.44411336585147865, -274.0450347767934431, -247.4583256500109485 ) ) ;
#60031=CARTESIAN_POINT ( 'NONE',  ( -71.74250447947856912, -195.9422791308210492, -360.7315132586310824 ) ) ;
#60032=CARTESIAN_POINT ( 'NONE',  ( -74.29123523874994817, -287.4770865509159989, -205.7239995025852579 ) ) ;
#60033=CARTESIAN_POINT ( 'NONE',  ( -93.44604478154516869, -298.3481232988896750, -217.9979353451291786 ) ) ;
#60034=CARTESIAN_POINT ( 'NONE',  ( -93.33852299750604686, -285.8699476186229163, -223.3691133751094640 ) ) ;
#60035=CARTESIAN_POINT ( 'NONE',  ( -73.99508255952055436, -276.5855836735034359, -337.8249430197521974 ) ) ;
#60036=CARTESIAN_POINT ( 'NONE',  ( 11.04819745993944480, -293.3530312216186644, -210.5286586992511104 ) ) ;
#60037=CARTESIAN_POINT ( 'NONE',  ( 35.51019780483819943, -285.4245286084055238, -249.3682159514878549 ) ) ;
#60038=CARTESIAN_POINT ( 'NONE',  ( 26.49658173305608599, -294.4523386142902837, -313.3776038982574619 ) ) ;
#60039=CARTESIAN_POINT ( 'NONE',  ( -91.69173430259594682, -291.5833271266084807, -221.5760195433436195 ) ) ;
#60042=CARTESIAN_POINT ( 'NONE',  ( -46.80064229259274811, -155.6065870647230440, -361.5538532369098448 ) ) ;
#60043=CARTESIAN_POINT ( 'NONE',  ( -100.4342404296290283, -286.6444321592520055, -227.3487617070399267 ) ) ;
#60044=CARTESIAN_POINT ( 'NONE',  ( -54.42813229853333468, -295.3380690714489560, -195.3538533559490702 ) ) ;
#60046=CARTESIAN_POINT ( 'NONE',  ( -65.44686644367027384, -282.3487444171194625, -338.0824241412300353 ) ) ;
#60047=CARTESIAN_POINT ( 'NONE',  ( -103.5897598217109845, -277.7068393319694337, -309.6694710042850716 ) ) ;
#60048=CARTESIAN_POINT ( 'NONE',  ( 36.29390644308807623, -283.7248411236676020, -283.7681907213568024 ) ) ;
#60049=CARTESIAN_POINT ( 'NONE',  ( 198.8865589563561969, 282.5583194059946663, -111.0619671203250221 ) ) ;
#60050=CARTESIAN_POINT ( 'NONE',  ( -34.51904984752484040, -281.5920573642800377, -346.7197385799287872 ) ) ;
#60051=CARTESIAN_POINT ( 'NONE',  ( -7.576410142704281370, -284.4644072194051887, -201.9076716328407031 ) ) ;
#60052=CARTESIAN_POINT ( 'NONE',  ( -75.82606838877276800, -275.4049506015747966, -205.0374892216299827 ) ) ;
#60053=CARTESIAN_POINT ( 'NONE',  ( -65.60230355358891075, -298.1646704465148332, -202.9865921156171851 ) ) ;
#60054=CARTESIAN_POINT ( 'NONE',  ( 29.19204912661200524, -291.8167075531522983, -239.0239114305246630 ) ) ;
#60055=CARTESIAN_POINT ( 'NONE',  ( -111.7267238633212685, -278.9585843775696503, -289.9110675159396919 ) ) ;
#60056=CARTESIAN_POINT ( 'NONE',  ( -11.25404169307784308, -276.7024905025317025, -338.5405435989334251 ) ) ;
#60057=CARTESIAN_POINT ( 'NONE',  ( -85.62432355126473738, -274.4814469709464788, -210.7768853010366286 ) ) ;
#60058=CARTESIAN_POINT ( 'NONE',  ( -94.98756247507560602, -276.7852675716887347, -320.9422119264992261 ) ) ;
#60059=CARTESIAN_POINT ( 'NONE',  ( -110.4262895430651383, -266.6388475384649155, -306.9518243255700440 ) ) ;
#60060=CARTESIAN_POINT ( 'NONE',  ( 32.88961892668422138, -273.8954262008013529, -296.8235451646469869 ) ) ;
#60061=CARTESIAN_POINT ( 'NONE',  ( -3.473499367217985245, -296.0391763085331718, -338.8705111685437146 ) ) ;
#60064=CARTESIAN_POINT ( 'NONE',  ( -91.88587535834876974, -284.9335426534595399, -319.3612137084307960 ) ) ;
#60065=CARTESIAN_POINT ( 'NONE',  ( -37.29210996487410057, -284.8116373413867564, -346.3606654925657722 ) ) ;
#60066=CARTESIAN_POINT ( 'NONE',  ( -62.59030357095917196, -285.0634391555424827, -201.7039252361940669 ) ) ;
#60068=CARTESIAN_POINT ( 'NONE',  ( -111.1506026067404775, -276.9846385056405893, -267.8610541376225456 ) ) ;
#60069=CARTESIAN_POINT ( 'NONE',  ( 18.55020681192583254, -284.0980071081172582, -319.2176448815467893 ) ) ;
#60070=CARTESIAN_POINT ( 'NONE',  ( -24.73896594693563245, -278.6957374422057683, -197.7534128682572430 ) ) ;
#60071=CARTESIAN_POINT ( 'NONE',  ( 5.588889963951293005, -277.5352739910390483, -329.8476334836412320 ) ) ;
#60073=CARTESIAN_POINT ( 'NONE',  ( -21.92715326418548472, -274.7474043191746773, -198.9441719092578751 ) ) ;
#60074=CARTESIAN_POINT ( 'NONE',  ( 37.71001984078320390, -282.5622074971882398, -286.8960834947649801 ) ) ;
#60075=CARTESIAN_POINT ( 'NONE',  ( -56.54735872776912231, -280.3035094294096439, -195.8033444586691019 ) ) ;
#60079=CARTESIAN_POINT ( 'NONE',  ( -10.45482138025249874, -288.2595266745221352, -199.4716193110464246 ) ) ;
#60080=CARTESIAN_POINT ( 'NONE',  ( -104.9074321217238293, -296.1248053154967579, -242.2991582027503625 ) ) ;
#60081=CARTESIAN_POINT ( 'NONE',  ( -40.61976135454321479, -291.3605619703167235, -193.5197871089743842 ) ) ;
#60082=CARTESIAN_POINT ( 'NONE',  ( 33.34041857083791172, -285.7581998457193322, -249.4660021938422005 ) ) ;
#60083=CARTESIAN_POINT ( 'NONE',  ( 3.930180888038329545, -287.0593590692782868, -331.3487941644067973 ) ) ;
#60084=CARTESIAN_POINT ( 'NONE',  ( -97.69112625662680216, -286.3363273289169797, -228.5647736578165166 ) ) ;
#60085=CARTESIAN_POINT ( 'NONE',  ( -111.7299583593154750, -276.6797949464423709, -260.4073693525061799 ) ) ;
#60086=CARTESIAN_POINT ( 'NONE',  ( -4.694487754694855575, -287.0291665085744057, -339.2274596313182542 ) ) ;
#60087=CARTESIAN_POINT ( 'NONE',  ( 23.89696215297717785, -288.9637462005171642, -227.0397144218443941 ) ) ;
#60088=CARTESIAN_POINT ( 'NONE',  ( -34.75601702405487003, -287.0195713830769932, -345.4833029360109435 ) ) ;
#60089=CARTESIAN_POINT ( 'NONE',  ( -16.05269163242585151, -283.7112393347064199, -340.4338413838113979 ) ) ;
#60090=CARTESIAN_POINT ( 'NONE',  ( -103.0207213337438645, -293.0377465651410489, -233.8057545256713468 ) ) ;
#60091=CARTESIAN_POINT ( 'NONE',  ( 82.14284478241719967, -300.0267218569679244, -193.4142195599097533 ) ) ;
#60093=CARTESIAN_POINT ( 'NONE',  ( -45.98979296249717663, -299.8634439075888167, -195.2976469253153766 ) ) ;
#60094=CARTESIAN_POINT ( 'NONE',  ( 17.18998019359640850, -280.0530794719977621, -221.5871744418945184 ) ) ;
#60095=CARTESIAN_POINT ( 'NONE',  ( 35.05055846913502648, -279.2993518184894128, -250.7067791094480640 ) ) ;
#60096=CARTESIAN_POINT ( 'NONE',  ( 33.26414128774135293, -293.1377728287725972, -300.8100319795473183 ) ) ;
#60097=CARTESIAN_POINT ( 'NONE',  ( -109.5181740824437213, -271.0052213271757182, -253.9742139346364240 ) ) ;
#60098=CARTESIAN_POINT ( 'NONE',  ( 37.02697664948645695, -273.5766100585297522, -266.0800591831813904 ) ) ;
#60099=CARTESIAN_POINT ( 'NONE',  ( -61.15724257057043900, -296.6829725821341412, -339.9424789945534826 ) ) ;
#60101=CARTESIAN_POINT ( 'NONE',  ( -103.7086846919696512, -271.6237411656142058, -232.3863919452905122 ) ) ;
#60102=CARTESIAN_POINT ( 'NONE',  ( -113.2233437110134133, -294.7300343687853683, -275.2515210284833529 ) ) ;
#60103=CARTESIAN_POINT ( 'NONE',  ( 20.63599331096736478, -294.3434659884822509, -225.0200663288813132 ) ) ;
#60105=CARTESIAN_POINT ( 'NONE',  ( 35.86962783226373119, -294.3601164790650841, -270.7506019270845741 ) ) ;
#60107=CARTESIAN_POINT ( 'NONE',  ( -69.07667481921521357, -283.6570217192106043, -202.0001651731305685 ) ) ;
#60108=CARTESIAN_POINT ( 'NONE',  ( 31.54005341148707942, -293.8755630787714495, -294.6848561595447791 ) ) ;
#60109=CARTESIAN_POINT ( 'NONE',  ( 13.68078880008794229, -282.3606358612337317, -328.1010212976989351 ) ) ;
#60110=CARTESIAN_POINT ( 'NONE',  ( -8.116955713747312728, -282.3520635717634377, -200.6676147848299081 ) ) ;
#60111=CARTESIAN_POINT ( 'NONE',  ( -106.6582305779312350, -284.6485668294866969, -236.8803339739678506 ) ) ;
#60112=CARTESIAN_POINT ( 'NONE',  ( -101.2647559451360451, -289.0747590808985024, -231.4526181405437910 ) ) ;
#60114=CARTESIAN_POINT ( 'NONE',  ( 34.94597919716335355, -280.3445120974340625, -294.9628594690515229 ) ) ;
#60115=CARTESIAN_POINT ( 'NONE',  ( -74.95823404620226427, -284.2245612456954404, -207.2244420008466079 ) ) ;
#60116=CARTESIAN_POINT ( 'NONE',  ( 28.63080754990374999, -286.9840178760042591, -309.4650914356356566 ) ) ;
#60118=CARTESIAN_POINT ( 'NONE',  ( -63.83738493670087877, -297.0034800188745407, -339.2949996874035605 ) ) ;
#60119=CARTESIAN_POINT ( 'NONE',  ( -99.16227662721641423, -279.3767094134034323, -315.2924080061521863 ) ) ;
#60120=CARTESIAN_POINT ( 'NONE',  ( 34.78778412533412023, -291.8540587322781903, -292.3492427028863290 ) ) ;
#60121=CARTESIAN_POINT ( 'NONE',  ( -32.95750494528525110, -279.7756245676312687, -197.4717064098965977 ) ) ;
#60122=CARTESIAN_POINT ( 'NONE',  ( -44.89915883971343646, -292.1257976000697454, -193.6799708958425583 ) ) ;
#60123=CARTESIAN_POINT ( 'NONE',  ( -112.7725404520761145, -282.5653148040115639, -275.5932424697898000 ) ) ;
#60124=CARTESIAN_POINT ( 'NONE',  ( -26.04539553192085677, -278.9084648984074875, -344.5055321279956502 ) ) ;
#60126=CARTESIAN_POINT ( 'NONE',  ( -12.94111007456871931, -293.7860022681561531, -339.4653921907678296 ) ) ;
#60127=CARTESIAN_POINT ( 'NONE',  ( -26.54324336545797181, -296.1871694351947326, -195.3647908593901263 ) ) ;
#60130=CARTESIAN_POINT ( 'NONE',  ( 32.60289517677492199, -283.1902606646293634, -244.1438174813643798 ) ) ;
#60131=CARTESIAN_POINT ( 'NONE',  ( -108.9462885836776849, -295.8676270808834943, -284.9414145441156734 ) ) ;
#60133=CARTESIAN_POINT ( 'NONE',  ( 10.64812456238590777, -272.1952119285918457, -210.2361428286349110 ) ) ;
#60134=CARTESIAN_POINT ( 'NONE',  ( 23.51123663286032084, -274.1216616260454089, -223.4240406178885792 ) ) ;
#60135=CARTESIAN_POINT ( 'NONE',  ( 39.08401493050234876, -288.8103014648780231, -265.8307958653457490 ) ) ;
#60136=CARTESIAN_POINT ( 'NONE',  ( -96.55985825834288505, -289.7884929461734487, -313.0484668365041330 ) ) ;
#60137=CARTESIAN_POINT ( 'NONE',  ( -92.74234073507324183, -280.7594970890079367, -221.7468872238774225 ) ) ;
#60138=CARTESIAN_POINT ( 'NONE',  ( -106.1696470976915379, -274.5059144561298581, -243.5901003498948114 ) ) ;
#60139=CARTESIAN_POINT ( 'NONE',  ( -95.09382783052089394, -277.9825165329937136, -225.0438502526426987 ) ) ;
#60141=CARTESIAN_POINT ( 'NONE',  ( -18.54791832922530759, -274.1209492767274583, -195.6348497170022540 ) ) ;
#60142=CARTESIAN_POINT ( 'NONE',  ( -86.90569370446500841, -293.2766925370726199, -214.7514189129017836 ) ) ;
#60145=CARTESIAN_POINT ( 'NONE',  ( -105.2045835335101742, -290.8387265926386931, -297.6726918875684191 ) ) ;
#60147=CARTESIAN_POINT ( 'NONE',  ( -50.33091995366235949, -290.0276058009588382, -195.7180630717236625 ) ) ;
#60148=CARTESIAN_POINT ( 'NONE',  ( -84.08511472884470095, -297.0558748295205760, -214.1957211572884603 ) ) ;
#60150=CARTESIAN_POINT ( 'NONE',  ( -105.8821533741155889, -291.6362835345876761, -304.0209006586660507 ) ) ;
#60151=CARTESIAN_POINT ( 'NONE',  ( -88.47809603358389552, -292.1948066931273615, -334.5364918783848793 ) ) ;
#60152=CARTESIAN_POINT ( 'NONE',  ( -30.38561211151381514, -288.1403637805460107, -195.7997077712545604 ) ) ;
#60153=CARTESIAN_POINT ( 'NONE',  ( -40.61072232799127590, -275.0931724856184815, -345.1357966490565445 ) ) ;
#60154=CARTESIAN_POINT ( 'NONE',  ( -4.698228753427344806, -276.4056702911311731, -203.4462169109697243 ) ) ;
#60155=CARTESIAN_POINT ( 'NONE',  ( -33.40836774472629855, -290.1818665307650349, -196.0123647669730076 ) ) ;
#60156=CARTESIAN_POINT ( 'NONE',  ( -38.18038781605122978, -281.9021564278876326, -194.6009563713172383 ) ) ;
#60157=ORIENTED_EDGE ( 'NONE', *, *, #45253, .F. ) ;
#60158=CARTESIAN_POINT ( 'NONE',  ( 30.42592407771797269, -281.2673194061783306, -297.7735563531068124 ) ) ;
#60159=CARTESIAN_POINT ( 'NONE',  ( -68.87565776265314810, -278.5367690266302247, -340.2832742911587616 ) ) ;
#60160=CARTESIAN_POINT ( 'NONE',  ( -76.56782556689915964, -282.3592685663999760, -336.2201920078268813 ) ) ;
#60161=CARTESIAN_POINT ( 'NONE',  ( -91.15551542514162975, -278.7352955428076484, -325.1794351223465469 ) ) ;
#60163=CARTESIAN_POINT ( 'NONE',  ( 15.53255164632434315, -276.3039156527190698, -215.3427460433160832 ) ) ;
#60164=CARTESIAN_POINT ( 'NONE',  ( -102.0172624299486870, -280.6233781216988064, -301.5434626090942061 ) ) ;
#60165=ORIENTED_EDGE ( 'NONE', *, *, #40970, .T. ) ;
#60167=CARTESIAN_POINT ( 'NONE',  ( -107.6904353227772901, -298.8914970349131295, -244.2101000726262612 ) ) ;
#60168=CARTESIAN_POINT ( 'NONE',  ( -26.41529573755634885, -289.9896548858116603, -342.9026579866572320 ) ) ;
#60169=CARTESIAN_POINT ( 'NONE',  ( -6.858512891713676396, -274.6701744502375959, -338.4979076164985372 ) ) ;
#60170=CARTESIAN_POINT ( 'NONE',  ( -7.299652639978720714, -290.4236878280474343, -340.1709421014539316 ) ) ;
#60171=CARTESIAN_POINT ( 'NONE',  ( -60.28309630248881490, -291.0954291505530591, -200.8991811606387898 ) ) ;
#60172=CARTESIAN_POINT ( 'NONE',  ( 10.18500508836902796, -287.9245591271960620, -330.9329336872447129 ) ) ;
#60174=CARTESIAN_POINT ( 'NONE',  ( -111.1083650188672465, -282.9809582191699633, -268.1431089663556691 ) ) ;
#60175=CARTESIAN_POINT ( 'NONE',  ( -83.29259632869344898, -291.5499034077038232, -328.6653255132981144 ) ) ;
#60176=CARTESIAN_POINT ( 'NONE',  ( -81.88239411230510711, -283.9124467166165005, -211.6513715178007544 ) ) ;
#60177=CARTESIAN_POINT ( 'NONE',  ( 20.89651535950630290, -282.2404050807076601, -225.5126246587260823 ) ) ;
#60178=CARTESIAN_POINT ( 'NONE',  ( 38.44464974120310785, -288.6507145488807851, -282.9013639530062960 ) ) ;
#60179=CARTESIAN_POINT ( 'NONE',  ( -109.1937588055996144, -279.2189980024490410, -257.1221563315460799 ) ) ;
#60180=CARTESIAN_POINT ( 'NONE',  ( -3.482959689871361952, -291.2840846420069170, -201.6327945492602396 ) ) ;
#60181=CARTESIAN_POINT ( 'NONE',  ( 14.13111054126479793, -287.5558469833566733, -213.2396894451537435 ) ) ;
#60182=CARTESIAN_POINT ( 'NONE',  ( 22.03867827054667927, -287.3866424217281406, -221.4377333414403211 ) ) ;
#60183=CARTESIAN_POINT ( 'NONE',  ( -109.8724925711547087, -284.6040743325395965, -279.0604625725920869 ) ) ;
#60186=CARTESIAN_POINT ( 'NONE',  ( -7.695715735095363108, -294.2969712121603720, -200.6231364379452771 ) ) ;
#60187=CARTESIAN_POINT ( 'NONE',  ( 23.62578397985801715, -292.8567483778737710, -316.5808557125232028 ) ) ;
#60188=CARTESIAN_POINT ( 'NONE',  ( 28.23587354593491838, -275.0529397128208302, -303.0789345688033904 ) ) ;
#60189=CARTESIAN_POINT ( 'NONE',  ( -82.90349917195925400, -296.7959896746002642, -208.3479271522658109 ) ) ;
#60190=CARTESIAN_POINT ( 'NONE',  ( 29.01046979033746354, -292.4632787213426468, -302.5426920484623565 ) ) ;
#60191=CARTESIAN_POINT ( 'NONE',  ( -80.29821245380310302, -295.7011154739013818, -210.0891339426439970 ) ) ;
#60192=CARTESIAN_POINT ( 'NONE',  ( -33.50293255450065288, -293.3065915030982183, -197.0519386510420361 ) ) ;
#60193=CARTESIAN_POINT ( 'NONE',  ( 33.60389554548378044, -294.3890767478114299, -251.8963263797545551 ) ) ;
#60195=CARTESIAN_POINT ( 'NONE',  ( -63.64898561860923820, -293.3941268106640905, -340.7738665185340210 ) ) ;
#60196=CARTESIAN_POINT ( 'NONE',  ( -110.4115052554880521, -298.7700237323742272, -253.3996235229373326 ) ) ;
#60197=CARTESIAN_POINT ( 'NONE',  ( 34.24321491439282283, -288.6974187575096948, -285.8798756206513758 ) ) ;
#60198=CARTESIAN_POINT ( 'NONE',  ( 17.71898388876078201, -278.2489727771535399, -321.8074772184902486 ) ) ;
#60199=CARTESIAN_POINT ( 'NONE',  ( 5.635761406164304432, -275.2788306918330932, -333.7720517227579080 ) ) ;
#60200=CARTESIAN_POINT ( 'NONE',  ( -32.68048206436853320, -273.4580076966628326, -193.5913184391545201 ) ) ;
#60201=CARTESIAN_POINT ( 'NONE',  ( 35.63767361693135882, -279.8226556343589664, -285.0991268998797068 ) ) ;
#60202=CARTESIAN_POINT ( 'NONE',  ( -107.9231706006774516, -276.5834894489800604, -299.0786464215859155 ) ) ;
#60204=CARTESIAN_POINT ( 'NONE',  ( -99.15710950568829674, -294.6894605470060355, -310.2048317315768031 ) ) ;
#60205=CARTESIAN_POINT ( 'NONE',  ( -112.3426406673569460, -274.5876385001751032, -267.6101980901121919 ) ) ;
#60206=CARTESIAN_POINT ( 'NONE',  ( -110.4436330666481183, -273.2034605540640086, -270.3693926218427919 ) ) ;
#60208=CARTESIAN_POINT ( 'NONE',  ( -71.40569764138540165, -289.6247439370711731, -203.1303845220607514 ) ) ;
#60209=CARTESIAN_POINT ( 'NONE',  ( -36.73393744560132745, -273.8933171697080979, -197.3512329030607759 ) ) ;
#60210=CARTESIAN_POINT ( 'NONE',  ( -20.49640521205113686, -288.8417219096920689, -345.5505711178771548 ) ) ;
#60211=CARTESIAN_POINT ( 'NONE',  ( -110.6607944582050607, -274.7645059448481675, -253.7979408056417867 ) ) ;
#60212=CARTESIAN_POINT ( 'NONE',  ( -108.6232173118451385, -294.2553407670069987, -293.3100488120630871 ) ) ;
#60213=CARTESIAN_POINT ( 'NONE',  ( 13.56614023886991482, -281.5579325093266903, -327.9866943903553533 ) ) ;
#60215=CARTESIAN_POINT ( 'NONE',  ( 36.03842940642930159, -279.3521498507132605, -254.7967583021844007 ) ) ;
#60217=CARTESIAN_POINT ( 'NONE',  ( -106.4113925128306732, -289.0181810814100913, -295.1906990955588981 ) ) ;
#60218=CARTESIAN_POINT ( 'NONE',  ( -110.7229842665056054, -282.5418030374244154, -281.9189072579788444 ) ) ;
#60221=CARTESIAN_POINT ( 'NONE',  ( -112.1188241497729052, -288.4696180742941465, -276.7763032269879773 ) ) ;
#60222=CARTESIAN_POINT ( 'NONE',  ( -72.25311772611807726, -275.1019721937089457, -205.4050948290368979 ) ) ;
#60223=CARTESIAN_POINT ( 'NONE',  ( -37.29898738808524428, -284.2566617434163732, -346.9770331353863639 ) ) ;
#60224=CARTESIAN_POINT ( 'NONE',  ( -43.89306941923850758, -272.0499383651509788, -195.0333546889487764 ) ) ;
#60225=CARTESIAN_POINT ( 'NONE',  ( -109.6122248940153412, -284.6879502116936465, -260.0668841569407164 ) ) ;
#60226=CARTESIAN_POINT ( 'NONE',  ( -1.164857568720132130, -277.9877671385102644, -334.5016323174721151 ) ) ;
#60227=CARTESIAN_POINT ( 'NONE',  ( -13.72362006023690739, -277.5405924947315270, -339.6587842107962274 ) ) ;
#60228=CARTESIAN_POINT ( 'NONE',  ( -78.05218136899647163, -285.5995863308420439, -333.3504612427573761 ) ) ;
#60232=CARTESIAN_POINT ( 'NONE',  ( -110.7796250023127413, -271.2951657040497935, -270.3451135339026905 ) ) ;
#60233=CARTESIAN_POINT ( 'NONE',  ( -79.47873886606210192, -295.4378054795741377, -334.8085381860692564 ) ) ;
#60234=CARTESIAN_POINT ( 'NONE',  ( -11.47513166114145555, -288.3706622350141515, -200.3413533579721957 ) ) ;
#60236=CARTESIAN_POINT ( 'NONE',  ( -117.3417001280813707, -275.0519495502701943, -270.3929463913696054 ) ) ;
#60237=CARTESIAN_POINT ( 'NONE',  ( -111.1467946632371167, -277.2102500921432124, -291.2009963621537167 ) ) ;
#60238=CARTESIAN_POINT ( 'NONE',  ( -106.5254538032993707, -289.3663254432653389, -238.2972757114068258 ) ) ;
#60239=CARTESIAN_POINT ( 'NONE',  ( -88.18673389239081928, -286.8445716099072911, -217.0179807214520906 ) ) ;
#60240=CARTESIAN_POINT ( 'NONE',  ( -103.0659069813546580, -280.7701125916995011, -236.2156670393682987 ) ) ;
#60241=CARTESIAN_POINT ( 'NONE',  ( -66.97741093497941733, -287.0965170357496845, -199.9315010687141410 ) ) ;
#60242=CARTESIAN_POINT ( 'NONE',  ( -7.680462126197816097, -284.6635433944708780, -339.2466143603145383 ) ) ;
#60243=CARTESIAN_POINT ( 'NONE',  ( -41.38232289034768030, -277.2683565401914620, -347.2682366834074514 ) ) ;
#60244=CARTESIAN_POINT ( 'NONE',  ( -35.74699414900050698, -296.0923198386323065, -195.7168507407495781 ) ) ;
#60245=CARTESIAN_POINT ( 'NONE',  ( -64.74034322147507226, -279.5375379301183330, -198.3443836432581406 ) ) ;
#60246=CARTESIAN_POINT ( 'NONE',  ( -102.4863371415567599, -298.9550658739826190, -234.3404230450854868 ) ) ;
#60249=CARTESIAN_POINT ( 'NONE',  ( -106.6662871844225293, -275.4805209788417528, -237.0123917617630980 ) ) ;
#60250=CARTESIAN_POINT ( 'NONE',  ( 74.14484272234649609, -297.5732043206075446, -194.6311733944271793 ) ) ;
#60252=CARTESIAN_POINT ( 'NONE',  ( -36.47172746892963602, -276.5486457846513417, -343.4299548495921499 ) ) ;
#60253=CARTESIAN_POINT ( 'NONE',  ( -44.02349718850356908, -275.1746640943948137, -193.9971262066018483 ) ) ;
#60254=CARTESIAN_POINT ( 'NONE',  ( 34.10982527358357430, -280.2524243061703260, -242.1535515154855602 ) ) ;
#60255=CARTESIAN_POINT ( 'NONE',  ( -53.60974514382409239, -291.0238988515947085, -342.5644747067432831 ) ) ;
#60256=CARTESIAN_POINT ( 'NONE',  ( -113.0888950202087671, -298.1886702332307095, -261.1377662027001634 ) ) ;
#60257=CARTESIAN_POINT ( 'NONE',  ( -61.45195794554442159, -296.5634570477599254, -343.1262905628850604 ) ) ;
#60258=CARTESIAN_POINT ( 'NONE',  ( 5.533705379969268812, -294.6339370999251628, -208.9646833250910731 ) ) ;
#60259=CARTESIAN_POINT ( 'NONE',  ( 36.13918433175174272, -279.3688671727073256, -256.1305820727551463 ) ) ;
#60260=CARTESIAN_POINT ( 'NONE',  ( -38.39838872102135525, -281.9589619749160079, -195.9159684115177242 ) ) ;
#60261=CARTESIAN_POINT ( 'NONE',  ( -97.24484975780916329, -295.2396601323035839, -226.1476748521939442 ) ) ;
#60262=CARTESIAN_POINT ( 'NONE',  ( -112.8041653303977228, -286.0139173228913023, -281.3093389377768858 ) ) ;
#60263=CARTESIAN_POINT ( 'NONE',  ( -96.02399003453884063, -288.8580964210298134, -314.3208354987219764 ) ) ;
#60264=CARTESIAN_POINT ( 'NONE',  ( -82.33048564276411696, -220.3546857680660196, -352.1821843074090452 ) ) ;
#60266=CARTESIAN_POINT ( 'NONE',  ( -36.11464794040890780, -287.6118182440138753, -346.7750486394689347 ) ) ;
#60267=CARTESIAN_POINT ( 'NONE',  ( 34.98072400148332406, -287.3529688752091147, -280.5295414112006824 ) ) ;
#60269=CARTESIAN_POINT ( 'NONE',  ( -71.58831737021651520, -284.5736588485382299, -338.9808069832134834 ) ) ;
#60270=CARTESIAN_POINT ( 'NONE',  ( -14.06271774850366540, -274.6959185158779064, -201.1500172392267132 ) ) ;
#60272=CARTESIAN_POINT ( 'NONE',  ( -34.95619835613400994, -291.0017558241210622, -193.6942414667640833 ) ) ;
#60273=CARTESIAN_POINT ( 'NONE',  ( 38.56855941326944048, -282.3584503686267340, -282.7294047206377172 ) ) ;
#60274=CARTESIAN_POINT ( 'NONE',  ( -9.135554972707513599, -281.9344844748413266, -199.4589238809577978 ) ) ;
#60275=CARTESIAN_POINT ( 'NONE',  ( -6.242801423961558349, -280.7829446263093587, -199.9295028669648104 ) ) ;
#60276=CARTESIAN_POINT ( 'NONE',  ( -68.52329096929361185, -279.6305960739908301, -204.3557515900368458 ) ) ;
#60277=CARTESIAN_POINT ( 'NONE',  ( 7.399455738971487229, -291.9094976428775681, -326.5171145203363494 ) ) ;
#60278=CARTESIAN_POINT ( 'NONE',  ( -95.01368496865339353, -240.5153381641504495, -341.9424385301951475 ) ) ;
#60280=CARTESIAN_POINT ( 'NONE',  ( 31.98586378361875759, -277.9220439906721936, -298.6721042649011224 ) ) ;
#60281=CARTESIAN_POINT ( 'NONE',  ( 188.9470303086956164, 271.4955109107032172, -139.4255392735582006 ) ) ;
#60282=CARTESIAN_POINT ( 'NONE',  ( 22.66595197881656176, -278.9633109306001870, -225.9444556358551779 ) ) ;
#60283=CARTESIAN_POINT ( 'NONE',  ( -37.14101340303343335, -297.4033232792091894, -197.2563542109352284 ) ) ;
#60284=CARTESIAN_POINT ( 'NONE',  ( 39.54515796689923235, -293.0950701058832237, -273.1785557095368517 ) ) ;
#60285=CARTESIAN_POINT ( 'NONE',  ( 154.0301839824525985, 204.4104515755834086, -214.4894503002514341 ) ) ;
#60286=CARTESIAN_POINT ( 'NONE',  ( -89.19502213159468340, -295.9146647860602570, -214.1660304428902180 ) ) ;
#60287=CARTESIAN_POINT ( 'NONE',  ( -71.56161040001792628, -287.9119001957585056, -335.7622317474711622 ) ) ;
#60288=CARTESIAN_POINT ( 'NONE',  ( -66.51713264913252033, -297.2987928475288868, -338.6228174872716181 ) ) ;
#60289=CARTESIAN_POINT ( 'NONE',  ( -38.65037451406145408, -287.3506136791974086, -196.8670521539149263 ) ) ;
#60291=CARTESIAN_POINT ( 'NONE',  ( 34.23906574697407734, -294.1393536794490728, -242.4831755626318284 ) ) ;
#60292=CARTESIAN_POINT ( 'NONE',  ( -95.96737624409604450, -284.4334301758705692, -313.9617893278019096 ) ) ;
#60293=CARTESIAN_POINT ( 'NONE',  ( -43.24377113548126772, -296.7742550785668527, -193.9329620962970750 ) ) ;
#60294=CARTESIAN_POINT ( 'NONE',  ( 22.07787360660950782, -293.6993719801215548, -221.6428146621456960 ) ) ;
#60295=CARTESIAN_POINT ( 'NONE',  ( 35.39237964450586560, -293.7262164888749112, -245.1144232785966324 ) ) ;
#60296=CARTESIAN_POINT ( 'NONE',  ( -63.81891468975411641, -289.5737869967754818, -338.4443925058523632 ) ) ;
#60299=CARTESIAN_POINT ( 'NONE',  ( -92.77545552695330855, -299.1287418647900722, -218.6376460912532593 ) ) ;
#60300=CARTESIAN_POINT ( 'NONE',  ( -78.61463545351449511, -272.3043817426019473, -205.8277659264548163 ) ) ;
#60301=CARTESIAN_POINT ( 'NONE',  ( 35.37191193793383093, -280.7310580270817582, -279.4994516254529913 ) ) ;
#60304=CARTESIAN_POINT ( 'NONE',  ( -4.027173323994664322, -276.1321952319327693, -339.7273831865137481 ) ) ;
#60306=CARTESIAN_POINT ( 'NONE',  ( -90.76177888933847271, -271.6785891852978807, -219.4237229612803617 ) ) ;
#60307=CARTESIAN_POINT ( 'NONE',  ( -110.8482623037358366, -280.5518020876081096, -259.6281508827213997 ) ) ;
#60308=CARTESIAN_POINT ( 'NONE',  ( 3.799293095429488787, -274.6313957641800698, -332.1533841260673512 ) ) ;
#60309=CARTESIAN_POINT ( 'NONE',  ( -92.15157593434433636, -298.4514762476190413, -221.5450548524433430 ) ) ;
#60310=CARTESIAN_POINT ( 'NONE',  ( -100.9279926597968284, -273.9908707611533032, -233.9246674225685467 ) ) ;
#60311=CARTESIAN_POINT ( 'NONE',  ( -111.1882564979777186, -297.9140611442166460, -289.2053987739818126 ) ) ;
#60312=CARTESIAN_POINT ( 'NONE',  ( 29.79652972768992925, -273.1219726962755203, -236.1432148959524397 ) ) ;
#60313=CARTESIAN_POINT ( 'NONE',  ( 10.36430436560265989, -295.0243135278672071, -325.7509167103522714 ) ) ;
#60314=CARTESIAN_POINT ( 'NONE',  ( -22.60503324030578298, -290.8192225406309035, -198.2625357183725043 ) ) ;
#60316=CARTESIAN_POINT ( 'NONE',  ( -67.67856717981702275, -277.9320459888386949, -341.0661489269728577 ) ) ;
#60317=CARTESIAN_POINT ( 'NONE',  ( -85.31176140418813247, -273.5343660305431399, -215.2676291830930779 ) ) ;
#60318=CARTESIAN_POINT ( 'NONE',  ( -41.55881333526495780, -281.7889124891074744, -346.8036464413556814 ) ) ;
#60319=CARTESIAN_POINT ( 'NONE',  ( 12.20692942455942642, -296.3652147582964176, -326.9541434600171783 ) ) ;
#60321=CARTESIAN_POINT ( 'NONE',  ( -110.4806728384389771, -283.7062194877621550, -273.6351884539421349 ) ) ;
#60322=CARTESIAN_POINT ( 'NONE',  ( -64.61140155105918836, -281.4071551656447241, -340.4206266324717376 ) ) ;
#60324=CARTESIAN_POINT ( 'NONE',  ( 35.28571244093176773, -274.2860847551515917, -282.5274744170075678 ) ) ;
#60325=CARTESIAN_POINT ( 'NONE',  ( 28.35337820628796379, -283.0699347400537249, -234.0724968215549211 ) ) ;
#60327=CARTESIAN_POINT ( 'NONE',  ( -112.3417001280813849, -275.0519495502701943, -270.3929463913730729 ) ) ;
#60328=CARTESIAN_POINT ( 'NONE',  ( -31.30293086102659572, -272.5270667090164238, -194.3876317211995399 ) ) ;
#60329=CARTESIAN_POINT ( 'NONE',  ( -90.02545959419016697, -279.7940334233845761, -324.0478788431071280 ) ) ;
#60331=CARTESIAN_POINT ( 'NONE',  ( -69.20824167837935192, -287.5564359016947265, -201.8354313154490001 ) ) ;
#60332=CARTESIAN_POINT ( 'NONE',  ( -110.1095955710663645, -288.7858685791759399, -252.1481033439261239 ) ) ;
#60334=CARTESIAN_POINT ( 'NONE',  ( -93.39552501683924390, -294.6771571863573627, -317.7630714065162465 ) ) ;
#60335=CARTESIAN_POINT ( 'NONE',  ( -66.84130882736201329, -287.5823003259767461, -338.5382902689954108 ) ) ;
#60336=CARTESIAN_POINT ( 'NONE',  ( 122.2132510144744231, 146.9671518294229884, -260.0597590233358574 ) ) ;
#60337=CARTESIAN_POINT ( 'NONE',  ( -66.32264754545623475, -295.6725654130979706, -201.1866621677464195 ) ) ;
#60338=CARTESIAN_POINT ( 'NONE',  ( 34.41381725791989510, -286.3646009679407030, -296.4734274704601376 ) ) ;
#60339=CARTESIAN_POINT ( 'NONE',  ( 36.50357674861623991, -283.1645900003296674, -271.3038625489959941 ) ) ;
#60340=CARTESIAN_POINT ( 'NONE',  ( -60.93856772378150310, -281.5940001801135963, -342.6459994047218629 ) ) ;
#60341=CARTESIAN_POINT ( 'NONE',  ( -110.1226431689860163, -290.4694564193342217, -276.6299076501842933 ) ) ;
#60342=CARTESIAN_POINT ( 'NONE',  ( 36.01798336709773452, -283.0614899264870132, -276.7846554825192698 ) ) ;
#60343=CARTESIAN_POINT ( 'NONE',  ( 18.62447054245579636, -283.0230564430576692, -317.5015775549690602 ) ) ;
#60344=CARTESIAN_POINT ( 'NONE',  ( -18.11904906768154433, -290.7854634704876275, -343.2232925734124933 ) ) ;
#60345=CARTESIAN_POINT ( 'NONE',  ( -114.3205561439199016, -272.8853797068901486, -270.3653521014397825 ) ) ;
#60347=CARTESIAN_POINT ( 'NONE',  ( -36.13483442274355895, -287.1170165586009375, -345.9243486391231386 ) ) ;
#60348=CARTESIAN_POINT ( 'NONE',  ( 39.13758532672542145, -275.6695467902663950, -279.7478967641140457 ) ) ;
#60349=CARTESIAN_POINT ( 'NONE',  ( 22.29299383757311404, -294.9154489403833281, -225.4662398637358649 ) ) ;
#60351=CARTESIAN_POINT ( 'NONE',  ( -106.6379572354042296, -286.6233781216988064, -303.7686719486574702 ) ) ;
#60352=CARTESIAN_POINT ( 'NONE',  ( 19.41871461515636454, -274.2343777766545259, -319.6582094377096155 ) ) ;
#60354=CARTESIAN_POINT ( 'NONE',  ( -112.0998145659246603, -295.1393257513942672, -255.5406399483490816 ) ) ;
#60355=CARTESIAN_POINT ( 'NONE',  ( -110.9184965776258025, -292.0693271024657633, -276.7188878244583066 ) ) ;
#60356=CARTESIAN_POINT ( 'NONE',  ( -54.22704220152846943, -273.1780817950580058, -199.2360317549228910 ) ) ;
#60357=CARTESIAN_POINT ( 'NONE',  ( -95.48576876399165769, -291.4401111558981370, -315.6581479910167900 ) ) ;
#60358=CARTESIAN_POINT ( 'NONE',  ( -36.21449393256687443, -293.0078456164562795, -197.1219812885336466 ) ) ;
#60359=CARTESIAN_POINT ( 'NONE',  ( -94.04569903959664146, -286.9784963019735073, -222.7940019961555436 ) ) ;
#60360=CARTESIAN_POINT ( 'NONE',  ( -70.65732792718868893, -293.0466318752395978, -201.5957543171193151 ) ) ;
#60361=CARTESIAN_POINT ( 'NONE',  ( -2.296752405834777910, -293.8212157918388243, -202.3379816396223134 ) ) ;
#60362=CARTESIAN_POINT ( 'NONE',  ( -10.49197628768942359, -294.5251384784609741, -338.2440490787099634 ) ) ;
#60363=CARTESIAN_POINT ( 'NONE',  ( 21.05686653724457358, -288.9044396604714393, -223.2811554807071843 ) ) ;
#60364=CARTESIAN_POINT ( 'NONE',  ( 31.07811630528027180, -282.1741526931518251, -305.6843217402886239 ) ) ;
#60365=CARTESIAN_POINT ( 'NONE',  ( -92.59277407053893683, -295.3487818320621727, -218.7422906775180138 ) ) ;
#60366=CARTESIAN_POINT ( 'NONE',  ( -102.5173452166442303, -284.9223813039850484, -229.3594681159061111 ) ) ;
#60367=CARTESIAN_POINT ( 'NONE',  ( 37.24682703375449222, -277.5838526821655705, -274.3765271141187441 ) ) ;
#60368=CARTESIAN_POINT ( 'NONE',  ( -66.73259335456813801, -282.2409125996175590, -337.6302913085501700 ) ) ;
#60369=CARTESIAN_POINT ( 'NONE',  ( 32.01976943006615528, -285.1782093018072715, -241.6948677089157798 ) ) ;
#60370=CARTESIAN_POINT ( 'NONE',  ( -28.76478048777695662, -275.0842267364463964, -345.6915977970836025 ) ) ;
#60372=CARTESIAN_POINT ( 'NONE',  ( -99.08639726049293017, -283.5193809196402412, -309.5145271514999195 ) ) ;
#60373=CARTESIAN_POINT ( 'NONE',  ( -111.3513979208076279, -280.0065270791583885, -250.5475088318775363 ) ) ;
#60374=CARTESIAN_POINT ( 'NONE',  ( 16.14386378315460746, -285.8476498692041332, -215.2964771897490266 ) ) ;
#60375=CARTESIAN_POINT ( 'NONE',  ( 33.32084354231822942, -295.6000628705302802, -292.3788139522815186 ) ) ;
#60376=CARTESIAN_POINT ( 'NONE',  ( 12.20010765938192598, -277.9761194971094938, -328.2580064537045814 ) ) ;
#60377=CARTESIAN_POINT ( 'NONE',  ( 23.23206548785715242, -276.2393255405116861, -223.6052599135365426 ) ) ;
#60378=CARTESIAN_POINT ( 'NONE',  ( -29.71553516543211160, -276.7863686243386496, -343.0125858697768422 ) ) ;
#60379=CARTESIAN_POINT ( 'NONE',  ( -101.4809558736667867, -299.0709051326151098, -231.7092294700630930 ) ) ;
#60380=CARTESIAN_POINT ( 'NONE',  ( 31.09153117124195731, -285.9510332009285776, -300.7702923337593006 ) ) ;
#60381=CARTESIAN_POINT ( 'NONE',  ( -84.65186673030201803, -291.2913822761420306, -330.1627423075444199 ) ) ;
#60382=CARTESIAN_POINT ( 'NONE',  ( 16.37632526507976038, -293.1865005834794147, -320.2469859380777848 ) ) ;
#60383=VERTEX_POINT ( 'NONE', #33074 ) ;
#60384=CARTESIAN_POINT ( 'NONE',  ( -52.36997697598155810, -291.5212123210685604, -198.8512544192556390 ) ) ;
#60386=CARTESIAN_POINT ( 'NONE',  ( -93.35757527685545654, -290.9139143489872481, -322.8181126954419256 ) ) ;
#60387=CARTESIAN_POINT ( 'NONE',  ( -100.9045231218293139, -279.6973710432708913, -234.2548830501746693 ) ) ;
#60389=CARTESIAN_POINT ( 'NONE',  ( -103.5758760150832245, -295.9787427896730492, -231.5973881383107198 ) ) ;
#60390=CARTESIAN_POINT ( 'NONE',  ( 32.77533583169434195, -288.6073964738947097, -301.9350638001409379 ) ) ;
#60391=CARTESIAN_POINT ( 'NONE',  ( -14.95434048996155596, -289.1032855208179058, -344.0684021427582593 ) ) ;
#60392=CARTESIAN_POINT ( 'NONE',  ( -110.0159010472469276, -284.9857822643265877, -262.7520650954139114 ) ) ;
#60393=CARTESIAN_POINT ( 'NONE',  ( 160.9517679153581753, 220.5049154629363102, -205.2241752943726283 ) ) ;
#60394=CARTESIAN_POINT ( 'NONE',  ( 83.03165031430961562, 83.43481754666375139, -300.8253819011565042 ) ) ;
#60395=CARTESIAN_POINT ( 'NONE',  ( -31.26167726347551223, -124.5763668223686835, -360.4898096339886706 ) ) ;
#60396=CARTESIAN_POINT ( 'NONE',  ( 17.54962551842718099, -275.4386829101774197, -318.7488484137036266 ) ) ;
#60397=CARTESIAN_POINT ( 'NONE',  ( -104.7207959087122333, -277.8588643062657866, -241.4771514175159552 ) ) ;
#60398=CARTESIAN_POINT ( 'NONE',  ( -83.56400558663789013, -273.1045818380775927, -208.7375805075950836 ) ) ;
#60399=CARTESIAN_POINT ( 'NONE',  ( -61.42094543554144792, -183.6680788050960302, -359.7854877795325592 ) ) ;
#60400=CARTESIAN_POINT ( 'NONE',  ( -62.26129571335676616, -276.0543080632585884, -342.7517924108050238 ) ) ;
#60402=CARTESIAN_POINT ( 'NONE',  ( -88.69987556725860145, -290.2895612397065292, -322.3257815257055654 ) ) ;
#60403=CARTESIAN_POINT ( 'NONE',  ( -91.52891105552558315, -298.1068700209668236, -215.8826360640291568 ) ) ;
#60404=CARTESIAN_POINT ( 'NONE',  ( 35.48715543661081995, -286.1029092815344370, -260.1297113658219473 ) ) ;
#60405=CARTESIAN_POINT ( 'NONE',  ( -76.38812534817202504, -274.1961429040649136, -204.0524023061860532 ) ) ;
#60406=CARTESIAN_POINT ( 'NONE',  ( -13.00624196479073191, -294.8937557311120941, -339.2386854501556854 ) ) ;
#60408=CARTESIAN_POINT ( 'NONE',  ( -34.32366762088548739, -278.9346321755835447, -345.8608244721069696 ) ) ;
#60409=CARTESIAN_POINT ( 'NONE',  ( 37.48705065781805246, -281.2844285935266839, -288.3110075054955814 ) ) ;
#60410=CARTESIAN_POINT ( 'NONE',  ( -79.24275955927753046, -280.5513155769745595, -210.2069220239609990 ) ) ;
#60411=CARTESIAN_POINT ( 'NONE',  ( -104.0748209470628751, -279.8357202494831881, -306.7020673000677675 ) ) ;
#60412=CARTESIAN_POINT ( 'NONE',  ( -107.8543212321808369, -271.3150099633287482, -248.7697013048455688 ) ) ;
#60414=CARTESIAN_POINT ( 'NONE',  ( -81.28957079212877090, -279.6026526462124480, -212.0088393225276207 ) ) ;
#60415=CARTESIAN_POINT ( 'NONE',  ( -99.44260204667226333, -273.9578133151052270, -225.0220549198278945 ) ) ;
#60416=CARTESIAN_POINT ( 'NONE',  ( -101.0343693207089757, -275.0841720468228573, -230.7600505899964958 ) ) ;
#60417=CARTESIAN_POINT ( 'NONE',  ( 16.52685502746049906, -274.8796504516705568, -324.6270949286655991 ) ) ;
#60419=CARTESIAN_POINT ( 'NONE',  ( -110.1325230367951633, -289.8461273554763125, -263.0059954806920928 ) ) ;
#60420=CARTESIAN_POINT ( 'NONE',  ( -113.4996134851687373, -283.7627389567925320, -281.3810550041005172 ) ) ;
#60421=CARTESIAN_POINT ( 'NONE',  ( 27.35534310518245604, -279.3072619147211526, -234.4130080426462825 ) ) ;
#60422=CARTESIAN_POINT ( 'NONE',  ( 36.29217619228348468, -280.1396761020107533, -271.3395607405268493 ) ) ;
#60423=CARTESIAN_POINT ( 'NONE',  ( -109.7608409365407169, -282.8555170516749513, -253.0789295292640304 ) ) ;
#60425=CARTESIAN_POINT ( 'NONE',  ( -73.73857301142604115, -291.5354534251313225, -335.9520805877830867 ) ) ;
#60426=CARTESIAN_POINT ( 'NONE',  ( 34.72118241597770094, -282.5735851738255633, -256.3640232395841849 ) ) ;
#60427=CARTESIAN_POINT ( 'NONE',  ( -49.16145522619329711, -155.7821930437820299, -366.3065075751858330 ) ) ;
#60428=CARTESIAN_POINT ( 'NONE',  ( 8.708969109741483194, -280.8325290187318615, -331.0717124137480596 ) ) ;
#60429=CARTESIAN_POINT ( 'NONE',  ( 24.86744961748311766, -296.1189489540585100, -312.2541047099462048 ) ) ;
#60430=CARTESIAN_POINT ( 'NONE',  ( -112.7090258089518642, -276.9197754974242685, -260.2797850532599568 ) ) ;
#60432=CARTESIAN_POINT ( 'NONE',  ( -96.17010578136677168, -278.5959504278434338, -313.7769278729720668 ) ) ;
#60433=CARTESIAN_POINT ( 'NONE',  ( -99.87933577908189875, -285.9889349030044627, -312.1566534656125214 ) ) ;
#60434=EDGE_CURVE ( 'NONE', #85445, #64930, #48199, .T. ) ;
#60435=EDGE_CURVE ( 'NONE', #9799, #31408, #56758, .T. ) ;
#60437=CARTESIAN_POINT ( 'NONE',  ( -19.74628914275245251, -294.1966729846561748, -196.8245676715132220 ) ) ;
#60438=CARTESIAN_POINT ( 'NONE',  ( 30.96558841734766787, -273.9582843052109524, -301.3306994664233684 ) ) ;
#60439=CARTESIAN_POINT ( 'NONE',  ( -18.21232186337783077, -285.4896455832965216, -195.8868729565939191 ) ) ;
#60440=CARTESIAN_POINT ( 'NONE',  ( -98.95633730131135053, -289.5104028974135986, -229.6471909792298050 ) ) ;
#60442=CARTESIAN_POINT ( 'NONE',  ( 17.79418301199583397, -274.9264242473320792, -318.9730797678557224 ) ) ;
#60443=CARTESIAN_POINT ( 'NONE',  ( -69.06636681671103872, -293.6134082483695238, -337.4899922149833742 ) ) ;
#60444=CARTESIAN_POINT ( 'NONE',  ( -106.4909477400585587, -291.5380246971271845, -295.2533865042721573 ) ) ;
#60447=CARTESIAN_POINT ( 'NONE',  ( 36.75339312711324169, -291.8018109438058900, -252.1231106745921977 ) ) ;
#60448=CARTESIAN_POINT ( 'NONE',  ( 34.15862023356043409, -288.9130158438732678, -252.0305447312458114 ) ) ;
#60449=CARTESIAN_POINT ( 'NONE',  ( -18.00412063822193787, -287.0460320457614216, -343.8460282081819628 ) ) ;
#60450=CARTESIAN_POINT ( 'NONE',  ( 11.51178007031639616, -288.1705333175712553, -215.2589294679796126 ) ) ;
#60452=CARTESIAN_POINT ( 'NONE',  ( 27.79726307608590119, -287.9020858653212258, -236.9400331837324529 ) ) ;
#60453=CARTESIAN_POINT ( 'NONE',  ( -66.26921147229691655, -297.4088277195949104, -339.9566630169336463 ) ) ;
#60455=CARTESIAN_POINT ( 'NONE',  ( -7.511988127940834481, -287.6395739469902537, -199.7484213841595704 ) ) ;
#60456=CARTESIAN_POINT ( 'NONE',  ( -59.27089505442766892, -275.4136943288603447, -342.6689640691782301 ) ) ;
#60457=CARTESIAN_POINT ( 'NONE',  ( -54.12250354081604087, -277.5950956193195225, -345.5432937424280340 ) ) ;
#60458=CARTESIAN_POINT ( 'NONE',  ( -69.94955670522723779, -279.3010920102036039, -200.6153053965879280 ) ) ;
#60459=CARTESIAN_POINT ( 'NONE',  ( -40.61477191305175438, -299.9907085589559870, -195.7752767430148140 ) ) ;
#60460=CARTESIAN_POINT ( 'NONE',  ( -99.75775605391878287, -283.1138997041495031, -228.7770271374152458 ) ) ;
#60462=CARTESIAN_POINT ( 'NONE',  ( -70.26716429366889827, -277.7531422142660062, -203.8129948819625383 ) ) ;
#60463=CARTESIAN_POINT ( 'NONE',  ( -99.76894582009430223, -281.9892592119396113, -312.0216398064575856 ) ) ;
#60465=CARTESIAN_POINT ( 'NONE',  ( 5.466182630333113579, -274.9638351995419043, -333.5290918702791600 ) ) ;
#60466=CARTESIAN_POINT ( 'NONE',  ( -53.28065189791139744, -296.7802625684204259, -342.3625864068833948 ) ) ;
#60467=CARTESIAN_POINT ( 'NONE',  ( 17.59520904227672844, -281.2098279357848583, -323.9479973300236111 ) ) ;
#60468=CARTESIAN_POINT ( 'NONE',  ( -95.48315923168142660, -298.1180668606017434, -225.8100260978594065 ) ) ;
#60469=CARTESIAN_POINT ( 'NONE',  ( -93.31347934851625325, -298.5835879158189528, -218.1258116344050393 ) ) ;
#60470=CARTESIAN_POINT ( 'NONE',  ( -74.28041603919683666, -273.2135572696998338, -207.3135097928088726 ) ) ;
#60471=CARTESIAN_POINT ( 'NONE',  ( 34.26366238025857314, -295.8400433992657668, -292.6696972553274918 ) ) ;
#60472=CARTESIAN_POINT ( 'NONE',  ( 33.85861635838831774, -287.3447010272027455, -240.9043486338368041 ) ) ;
#60473=CARTESIAN_POINT ( 'NONE',  ( -109.1729696449280027, -276.9344563478626355, -246.7520387146150256 ) ) ;
#60474=CARTESIAN_POINT ( 'NONE',  ( -113.8138157160755810, -290.2673993167886124, -279.8021662227334900 ) ) ;
#60475=CARTESIAN_POINT ( 'NONE',  ( -18.42424667314170961, -287.8612621802606100, -341.1637006831845156 ) ) ;
#60476=CARTESIAN_POINT ( 'NONE',  ( 3.085500285982334834, -290.5944646524255859, -207.1280172241680191 ) ) ;
#60478=CARTESIAN_POINT ( 'NONE',  ( -32.04911714649202992, -124.5213432794980974, -365.6788127701597659 ) ) ;
#60479=CARTESIAN_POINT ( 'NONE',  ( 34.06949131471166936, -287.2640519193242881, -285.8609546571488522 ) ) ;
#60481=CARTESIAN_POINT ( 'NONE',  ( -79.02188655731423239, -284.5408484617651084, -334.8249238877208427 ) ) ;
#60482=CARTESIAN_POINT ( 'NONE',  ( -30.70562566366761814, -291.1927188127653494, -193.8311861543629391 ) ) ;
#60483=CARTESIAN_POINT ( 'NONE',  ( 30.64661842002393399, -283.3224618116423130, -305.4451145117475335 ) ) ;
#60484=CARTESIAN_POINT ( 'NONE',  ( -65.31765963758300586, -283.2615883188624366, -337.8013115896732756 ) ) ;
#60485=CARTESIAN_POINT ( 'NONE',  ( -114.2338118077027218, -296.4898922198067908, -275.3393729434181978 ) ) ;
#60486=CARTESIAN_POINT ( 'NONE',  ( 32.52544030834806676, -276.5648781178616105, -247.3978271721397846 ) ) ;
#60487=CARTESIAN_POINT ( 'NONE',  ( 35.25317974580958236, -291.3474700368367394, -252.9331715136766547 ) ) ;
#60488=CARTESIAN_POINT ( 'NONE',  ( 30.54791512914200524, -273.9736478377423623, -242.3326003459168874 ) ) ;
#60491=CARTESIAN_POINT ( 'NONE',  ( 3.211412914798389640, -288.5218311975210099, -207.9370904057302596 ) ) ;
#60492=CARTESIAN_POINT ( 'NONE',  ( -27.77271544623243571, -296.0131518667982391, -346.5057671648525002 ) ) ;
#60493=CARTESIAN_POINT ( 'NONE',  ( -101.8572910434111805, -284.7344842269143896, -304.8436945102615141 ) ) ;
#60494=CARTESIAN_POINT ( 'NONE',  ( 30.32996426721521033, -275.0820113036388079, -306.7137162957004648 ) ) ;
#60495=CARTESIAN_POINT ( 'NONE',  ( 39.33879950311789031, -294.1311753769712141, -264.5806541041093851 ) ) ;
#60496=CARTESIAN_POINT ( 'NONE',  ( 36.29816829439095471, -285.9188744056791620, -288.2336879446320381 ) ) ;
#60497=AXIS2_PLACEMENT_3D ( 'NONE', #21337, #49743, #63989 ) ;
#60498=CARTESIAN_POINT ( 'NONE',  ( 1.762351128586354454, -294.8772926592548060, -336.6681120844520478 ) ) ;
#60499=CARTESIAN_POINT ( 'NONE',  ( -86.74056144057361450, -290.0948930024592300, -324.2055395784946654 ) ) ;
#60502=CARTESIAN_POINT ( 'NONE',  ( -88.12805157378475940, -229.8124237020200837, -344.5111176630173304 ) ) ;
#60504=CARTESIAN_POINT ( 'NONE',  ( -66.93817202083411644, -287.1913513824442248, -200.0279351660444718 ) ) ;
#60505=CARTESIAN_POINT ( 'NONE',  ( 40.65961533371913106, -278.8380690714489560, -252.5904736702033802 ) ) ;
#60507=CARTESIAN_POINT ( 'NONE',  ( -42.97031193815468697, -282.0450455850189542, -343.5041302086287374 ) ) ;
#60508=CARTESIAN_POINT ( 'NONE',  ( -87.08476619684397235, -277.3894779953670309, -329.1792417500458328 ) ) ;
#60509=CARTESIAN_POINT ( 'NONE',  ( 37.53760656589423661, -283.5645577198256433, -271.3122625095609237 ) ) ;
#60510=CARTESIAN_POINT ( 'NONE',  ( -20.05301036732419462, -109.6085418338271325, -361.2089085121472181 ) ) ;
#60511=CARTESIAN_POINT ( 'NONE',  ( -65.05553085888470832, -281.9819505822722476, -341.5830082621079669 ) ) ;
#60512=CARTESIAN_POINT ( 'NONE',  ( 37.32636870389302430, -285.5455533740810097, -268.2914573979493866 ) ) ;
#60513=CARTESIAN_POINT ( 'NONE',  ( -67.07311219661875157, -275.5269561293563925, -200.6736110778851128 ) ) ;
#60514=CARTESIAN_POINT ( 'NONE',  ( -63.58524729297759848, -295.8958775393900851, -338.6002356537047149 ) ) ;
#60515=CARTESIAN_POINT ( 'NONE',  ( 33.78970379422997183, -291.9946186084454212, -251.8795905768408829 ) ) ;
#60516=CARTESIAN_POINT ( 'NONE',  ( -108.4216000602299061, -279.5769834915836896, -241.0189876586613593 ) ) ;
#60517=CARTESIAN_POINT ( 'NONE',  ( -24.32960295472098267, -276.8815240205642567, -342.2435184127699586 ) ) ;
#60518=CARTESIAN_POINT ( 'NONE',  ( 37.28786742031591217, -274.6949080942545720, -288.0789004629479564 ) ) ;
#60520=CARTESIAN_POINT ( 'NONE',  ( 23.05401909177898645, -272.9452268401891502, -225.8724155096909101 ) ) ;
#60521=CARTESIAN_POINT ( 'NONE',  ( 33.90865761725102345, -295.3298246709218802, -297.9653352845036807 ) ) ;
#60524=CARTESIAN_POINT ( 'NONE',  ( -110.3034882577515106, -285.7320522267272622, -262.7314890404674088 ) ) ;
#60525=CARTESIAN_POINT ( 'NONE',  ( -31.68900807216368065, -284.7418921529511522, -346.1503361395804177 ) ) ;
#60526=CARTESIAN_POINT ( 'NONE',  ( -42.67329689383888081, -285.3317287527656845, -197.4412272059102236 ) ) ;
#60527=CARTESIAN_POINT ( 'NONE',  ( -73.24887588890946688, -275.9365228485140165, -334.8513535008983126 ) ) ;
#60528=CARTESIAN_POINT ( 'NONE',  ( 16.74174465225318897, -284.1330837846441568, -321.2865270618526665 ) ) ;
#60529=CARTESIAN_POINT ( 'NONE',  ( -104.9148116344691317, -276.6388864316090803, -299.8928449021976803 ) ) ;
#60530=CARTESIAN_POINT ( 'NONE',  ( 1.044953632588694781, -277.6067450453736569, -332.8762833897277460 ) ) ;
#60532=CARTESIAN_POINT ( 'NONE',  ( -103.2782961899313108, -279.8716610418654795, -230.8048308979910246 ) ) ;
#60533=CARTESIAN_POINT ( 'NONE',  ( 33.11407624544944639, -281.6499648306585186, -239.4497854544152915 ) ) ;
#60537=CARTESIAN_POINT ( 'NONE',  ( 37.45942772654314723, -289.5697300886031940, -282.7263006920437647 ) ) ;
#60538=CARTESIAN_POINT ( 'NONE',  ( -96.22421295610264735, -296.3568010194084081, -226.9181863685478220 ) ) ;
#60539=CARTESIAN_POINT ( 'NONE',  ( -70.60250078612546076, -288.8277924496885021, -339.7083474993643222 ) ) ;
#60540=CARTESIAN_POINT ( 'NONE',  ( 33.64818717020367700, -285.5182193394552428, -249.3781218782071392 ) ) ;
#60541=CARTESIAN_POINT ( 'NONE',  ( 36.03794416984193560, -286.2078452335103975, -276.5488024868615753 ) ) ;
#60542=CARTESIAN_POINT ( 'NONE',  ( -110.4232096375316701, -288.6386401632899492, -282.1485428781422797 ) ) ;
#60543=CARTESIAN_POINT ( 'NONE',  ( -54.86593816862129813, -287.0270325313683770, -199.0341927750866375 ) ) ;
#60544=CARTESIAN_POINT ( 'NONE',  ( -56.43998825413677167, -275.2979696075724405, -342.9423686592047034 ) ) ;
#60545=CARTESIAN_POINT ( 'NONE',  ( -2.188096729433388177, -286.9945401694358225, -337.9678083718283688 ) ) ;
#60546=CARTESIAN_POINT ( 'NONE',  ( -5.643018050268392649, -288.4691924920522865, -202.3891075114036084 ) ) ;
#60547=CARTESIAN_POINT ( 'NONE',  ( -45.84430722351293497, -287.1594166389476186, -345.0972097400667167 ) ) ;
#60548=CARTESIAN_POINT ( 'NONE',  ( -36.17780863960586402, -283.9784588265530942, -343.5871639324492435 ) ) ;
#60549=CARTESIAN_POINT ( 'NONE',  ( -104.8553635282622025, -292.1162448210491220, -303.5237687887135962 ) ) ;
#60553=CARTESIAN_POINT ( 'NONE',  ( -99.57872012755365176, -299.0489784469172037, -227.4913452869886612 ) ) ;
#60554=CARTESIAN_POINT ( 'NONE',  ( -46.46648324612441883, -279.1306978598997262, -197.7196833028347953 ) ) ;
#60555=CARTESIAN_POINT ( 'NONE',  ( 36.30282800205460347, -279.3688671705141928, -256.0988322388138272 ) ) ;
#60556=CARTESIAN_POINT ( 'NONE',  ( 39.55003942692350449, -292.7488089563902918, -270.3202706118128731 ) ) ;
#60557=CARTESIAN_POINT ( 'NONE',  ( -92.76226730721126046, -271.4833460967124097, -221.3046734687274864 ) ) ;
#60558=CARTESIAN_POINT ( 'NONE',  ( 24.53666851091549361, -280.7829715364869116, -310.1070178101709303 ) ) ;
#60559=CARTESIAN_POINT ( 'NONE',  ( -37.84353444839104696, -275.1382964924279690, -344.8121285912944245 ) ) ;
#60560=CARTESIAN_POINT ( 'NONE',  ( -88.83551304192404530, -297.1087385594521493, -322.8695417592547301 ) ) ;
#60562=CARTESIAN_POINT ( 'NONE',  ( -15.04264616131752064, -296.8064226372752046, -194.0600888125450467 ) ) ;
#60563=CARTESIAN_POINT ( 'NONE',  ( -44.71984174023356218, -293.3840368724249288, -346.0414434558113044 ) ) ;
#60564=CARTESIAN_POINT ( 'NONE',  ( 26.73879230165602650, -294.4848933392556773, -234.0761079441385277 ) ) ;
#60566=CARTESIAN_POINT ( 'NONE',  ( 35.58620969732011474, -294.4318767629111449, -276.2024958275785593 ) ) ;
#60570=CARTESIAN_POINT ( 'NONE',  ( -63.36810191647938950, -281.4097083275216278, -341.0791016373691491 ) ) ;
#60571=CARTESIAN_POINT ( 'NONE',  ( 17.08056822218696880, -294.2483305425531626, -319.0340156440103669 ) ) ;
#60572=CARTESIAN_POINT ( 'NONE',  ( 2.094138187946521512, -282.5393889787492299, -336.4959397961259242 ) ) ;
#60573=CARTESIAN_POINT ( 'NONE',  ( 36.57086068559772940, -283.2715198885970267, -254.6070352888611978 ) ) ;
#60575=CARTESIAN_POINT ( 'NONE',  ( -40.81126966245135179, -285.6764845111841851, -193.4083124510580092 ) ) ;
#60576=CARTESIAN_POINT ( 'NONE',  ( -80.56948442246236652, -289.4648332325664910, -209.2125360946509716 ) ) ;
#60577=CARTESIAN_POINT ( 'NONE',  ( 26.13429704387030483, -280.5945619526020778, -312.7109176932845571 ) ) ;
#60578=CARTESIAN_POINT ( 'NONE',  ( 0.4364395159697663229, -285.2513440326130763, -207.2616693030522868 ) ) ;
#60579=CARTESIAN_POINT ( 'NONE',  ( -9.687671272622218055, -287.6195282366902575, -341.8925600049396394 ) ) ;
#60581=CARTESIAN_POINT ( 'NONE',  ( -35.61165264579608447, -296.6302519773774407, -344.1534726132274500 ) ) ;
#60582=CARTESIAN_POINT ( 'NONE',  ( -9.410176537001710528, -278.1194006394584335, -341.4838027099662554 ) ) ;
#60583=CARTESIAN_POINT ( 'NONE',  ( -32.15151727363704737, -293.0071247618849384, -345.5503410003860267 ) ) ;
#60584=CARTESIAN_POINT ( 'NONE',  ( -83.44780380070754688, -279.0667575865829235, -213.6713462875808602 ) ) ;
#60585=CARTESIAN_POINT ( 'NONE',  ( 17.48811442845540043, -292.9756695827549038, -216.2241180179798050 ) ) ;
#60586=CARTESIAN_POINT ( 'NONE',  ( -96.43857024671335409, -283.2744289753583757, -223.2774249978915861 ) ) ;
#60587=CARTESIAN_POINT ( 'NONE',  ( -17.85241623260458610, -278.8009893531771013, -342.7846532393796224 ) ) ;
#60588=CARTESIAN_POINT ( 'NONE',  ( -7.904696112840743361, -293.7154938753760121, -337.4334528087462672 ) ) ;
#60589=CARTESIAN_POINT ( 'NONE',  ( -90.84577750382673855, -271.2949341975801758, -217.5658328722028898 ) ) ;
#60592=CARTESIAN_POINT ( 'NONE',  ( -3.626719288247383322, -282.4791681233259624, -203.7500174577812118 ) ) ;
#60593=CARTESIAN_POINT ( 'NONE',  ( -15.58047257130720276, -294.2705986754926926, -340.1598514669502720 ) ) ;
#60595=CARTESIAN_POINT ( 'NONE',  ( -106.6379572354042296, -270.4809262143061233, -236.9535640164627353 ) ) ;
#60596=CARTESIAN_POINT ( 'NONE',  ( -54.53078975202447509, -296.8952345963784865, -195.5456422427284906 ) ) ;
#60597=CARTESIAN_POINT ( 'NONE',  ( 5.296460762930212951, -289.8033955440743625, -333.8850151207809063 ) ) ;
#60598=CARTESIAN_POINT ( 'NONE',  ( -23.78725754470517018, -288.7075739331700674, -342.1434033988199985 ) ) ;
#60599=CARTESIAN_POINT ( 'NONE',  ( -24.77703228413670189, -281.7354919470448067, -197.7468158597859826 ) ) ;
#60600=CARTESIAN_POINT ( 'NONE',  ( -80.33463390192298448, -299.2208312046917058, -210.1151085145808679 ) ) ;
#60601=CARTESIAN_POINT ( 'NONE',  ( -16.79594119653510376, -279.1184445013944924, -199.8983455861094001 ) ) ;
#60603=CARTESIAN_POINT ( 'NONE',  ( -57.38012185026543932, -297.4672460197297141, -195.9808532764782001 ) ) ;
#60604=CARTESIAN_POINT ( 'NONE',  ( -91.82957718802086333, -293.1875909031014658, -219.6235749595483355 ) ) ;
#60606=CARTESIAN_POINT ( 'NONE',  ( -99.80300282278302859, -291.7259055380560540, -232.3811451849066430 ) ) ;
#60608=CARTESIAN_POINT ( 'NONE',  ( 20.38496360662549733, -291.0192152930006841, -221.2705473242575067 ) ) ;
#60609=CARTESIAN_POINT ( 'NONE',  ( -106.3624677003556229, -272.3781973416595292, -246.4002731446144026 ) ) ;
#60612=CARTESIAN_POINT ( 'NONE',  ( -113.6961392413176952, -292.0611784968479014, -271.2402657328650548 ) ) ;
#60613=CARTESIAN_POINT ( 'NONE',  ( -72.08107566293803359, -288.1233781216987495, -198.2974183793908196 ) ) ;
#60614=CARTESIAN_POINT ( 'NONE',  ( 10.17546534086699417, -288.7094029349109405, -212.5498093207402803 ) ) ;
#60615=CARTESIAN_POINT ( 'NONE',  ( 12.79320847787570692, -272.7529408060775040, -214.7348697397721935 ) ) ;
#60616=CARTESIAN_POINT ( 'NONE',  ( 27.88677906717059329, -276.9905502895525728, -234.3851046867563070 ) ) ;
#60617=CARTESIAN_POINT ( 'NONE',  ( 15.92264603349519092, -290.8935415500233717, -218.2851128831837855 ) ) ;
#60618=CARTESIAN_POINT ( 'NONE',  ( -50.74476704198991683, -281.7431036626027208, -195.7912629784086391 ) ) ;
#60620=CARTESIAN_POINT ( 'NONE',  ( 15.89440995821195912, -281.6216598381349741, -320.5321354122337993 ) ) ;
#60621=CARTESIAN_POINT ( 'NONE',  ( -64.97082253458765422, -278.4842878120849150, -341.9582392192971270 ) ) ;
#60622=CARTESIAN_POINT ( 'NONE',  ( 36.22271522649956665, -280.0772904032810402, -248.9532191077369419 ) ) ;
#60623=CARTESIAN_POINT ( 'NONE',  ( -84.15502384080009790, -218.1365120809277869, -349.3283341728729852 ) ) ;
#60624=CARTESIAN_POINT ( 'NONE',  ( 36.27125077342100212, -276.7678838039670950, -292.1779974731985021 ) ) ;
#60626=CARTESIAN_POINT ( 'NONE',  ( -5.422082409212579890, -275.9846430709311562, -201.0513368564109840 ) ) ;
#60627=CARTESIAN_POINT ( 'NONE',  ( -107.3417001280813565, -275.0519495502701943, -270.3929463913696054 ) ) ;
#60628=EDGE_LOOP ( 'NONE', ( #67269, #54080, #40528, #11678 ) ) ;
#60631=CARTESIAN_POINT ( 'NONE',  ( -63.92019387127945151, -290.4866310520984598, -338.7368989656019949 ) ) ;
#60632=CARTESIAN_POINT ( 'NONE',  ( -79.95356955140357513, -291.3797356019202880, -333.3389183249099119 ) ) ;
#60633=CARTESIAN_POINT ( 'NONE',  ( -5.990401590645244134, -291.8240484974339211, -204.3095332323871673 ) ) ;
#60634=CARTESIAN_POINT ( 'NONE',  ( 0.2591966413363832600, -286.0466692120098742, -203.2215746124874443 ) ) ;
#60636=CARTESIAN_POINT ( 'NONE',  ( -34.83960815200947536, -281.4201037312869289, -344.1312666608919244 ) ) ;
#60637=CARTESIAN_POINT ( 'NONE',  ( 30.56438278280192122, -289.8109883746771516, -300.4825694039474797 ) ) ;
#60638=CARTESIAN_POINT ( 'NONE',  ( -15.94955111743373166, -281.2502617265599838, -340.8812123653286790 ) ) ;
#60639=CARTESIAN_POINT ( 'NONE',  ( 13.66539583930616608, -282.0998886256161882, -217.3797276448290461 ) ) ;
#60640=CARTESIAN_POINT ( 'NONE',  ( 35.62163048327094828, -288.1904000803211829, -246.3338642848808888 ) ) ;
#60641=CARTESIAN_POINT ( 'NONE',  ( -109.5519304134525811, -278.8979240095968635, -281.4818681303011658 ) ) ;
#60642=CARTESIAN_POINT ( 'NONE',  ( -34.95731865161447871, -290.8763717674611371, -193.7822246757606308 ) ) ;
#60643=CARTESIAN_POINT ( 'NONE',  ( -3.569570110258568629, -287.2893896940269087, -201.3277687750509415 ) ) ;
#60644=CARTESIAN_POINT ( 'NONE',  ( -21.00315195154998094, -286.7487581783250334, -195.1774844807272302 ) ) ;
#60645=CARTESIAN_POINT ( 'NONE',  ( -45.63736041356587947, -283.3267614128931200, -342.9392243435241880 ) ) ;
#60648=CARTESIAN_POINT ( 'NONE',  ( -30.82747045714212675, -293.9939348471471590, -194.8249673091273166 ) ) ;
#60649=CARTESIAN_POINT ( 'NONE',  ( 36.23454281326554849, -291.9718552417300543, -249.3411071071053868 ) ) ;
#60650=CARTESIAN_POINT ( 'NONE',  ( 11.89706470054795240, -275.4068562313950679, -324.6420278999225957 ) ) ;
#60652=CARTESIAN_POINT ( 'NONE',  ( -113.6725936094580334, -296.0174851816216801, -261.0386994760402786 ) ) ;
#60653=CARTESIAN_POINT ( 'NONE',  ( 2.632699257351296396, -291.0783868558146423, -208.3914105678887836 ) ) ;
#60654=CARTESIAN_POINT ( 'NONE',  ( -111.1111930172054656, -294.7060404322562022, -276.9681024101976163 ) ) ;
#60655=CARTESIAN_POINT ( 'NONE',  ( -84.09370055757085538, -292.5976536416226281, -213.7803707316678867 ) ) ;
#60656=CARTESIAN_POINT ( 'NONE',  ( -7.155473100384013740, -293.5374214434013993, -203.5552965871385709 ) ) ;
#60658=CARTESIAN_POINT ( 'NONE',  ( 19.95329039137341454, -292.2238954011986607, -319.0161536000966862 ) ) ;
#60659=CARTESIAN_POINT ( 'NONE',  ( -111.9868657989353125, -298.4522530729223035, -278.1542108845709436 ) ) ;
#60660=CARTESIAN_POINT ( 'NONE',  ( 21.36927718300752588, -289.1058965491647541, -314.1591588142248952 ) ) ;
#60661=CARTESIAN_POINT ( 'NONE',  ( -42.66428027571386394, -279.0988923518869456, -345.5281116963840873 ) ) ;
#60662=CARTESIAN_POINT ( 'NONE',  ( -84.63336088318990846, -276.4818810966186788, -330.6905201133657215 ) ) ;
#60663=CARTESIAN_POINT ( 'NONE',  ( -70.08082301010752246, -272.9807356821661415, -200.7661047113763857 ) ) ;
#60664=CARTESIAN_POINT ( 'NONE',  ( -1.761476353488416358, -280.6567830265450993, -335.7619383418527832 ) ) ;
#60665=CARTESIAN_POINT ( 'NONE',  ( -90.78265971792666278, -276.1943246467036488, -324.7535736170409564 ) ) ;
#60667=CARTESIAN_POINT ( 'NONE',  ( -106.4566453505326251, -294.9045789936268989, -295.4982061777914737 ) ) ;
#60669=CARTESIAN_POINT ( 'NONE',  ( -106.4054009945861168, -273.5217733763906836, -246.4007780283252487 ) ) ;
#60671=CARTESIAN_POINT ( 'NONE',  ( -96.87598455088541982, -287.9419036202641564, -316.5571760960855272 ) ) ;
#60672=CARTESIAN_POINT ( 'NONE',  ( 32.06247581584992901, -275.0832630219227894, -247.5697406013929083 ) ) ;
#60673=CARTESIAN_POINT ( 'NONE',  ( -1.800723475625440217, -288.5944098374249052, -338.6680647639055906 ) ) ;
#60674=CARTESIAN_POINT ( 'NONE',  ( -33.46609864687144409, -300.0803253697694117, -195.0046094052071055 ) ) ;
#60675=CARTESIAN_POINT ( 'NONE',  ( -111.9287426032308872, -294.4660598388139192, -277.0385069591173419 ) ) ;
#60676=CARTESIAN_POINT ( 'NONE',  ( -65.20318946247230940, -282.6042898598732336, -341.9846234622050360 ) ) ;
#60678=CARTESIAN_POINT ( 'NONE',  ( -40.69529884830035371, -281.0941508278524452, -345.2987983457802557 ) ) ;
#60680=CARTESIAN_POINT ( 'NONE',  ( -110.7342668994143224, -289.3363972647138098, -271.1745344386482657 ) ) ;
#60681=CARTESIAN_POINT ( 'NONE',  ( -70.79237701084589673, -281.6377308945866389, -336.6468801284265169 ) ) ;
#60684=CARTESIAN_POINT ( 'NONE',  ( -78.32737713689711256, -289.5005245642581144, -207.5504904803935631 ) ) ;
#60685=CARTESIAN_POINT ( 'NONE',  ( -90.71196182556371923, -274.7983362236321909, -219.5260891830804155 ) ) ;
#60686=CARTESIAN_POINT ( 'NONE',  ( 13.42915876502997286, -283.5655176203714518, -327.7931232356754094 ) ) ;
#60687=CARTESIAN_POINT ( 'NONE',  ( -41.09628269797579492, -272.0852301156956514, -194.8431711031664406 ) ) ;
#60688=CARTESIAN_POINT ( 'NONE',  ( -109.8727451829732757, -284.4374211599986211, -279.0583553752116472 ) ) ;
#60689=CARTESIAN_POINT ( 'NONE',  ( 35.94243518132184789, -277.0650297401658122, -277.0551771541302628 ) ) ;
#60690=CARTESIAN_POINT ( 'NONE',  ( -45.91689934074382506, -277.9663590566264020, -343.0690483393344721 ) ) ;
#60691=CARTESIAN_POINT ( 'NONE',  ( 29.31168984804137523, -284.0073380426781000, -304.7460892699423312 ) ) ;
#60694=CARTESIAN_POINT ( 'NONE',  ( 28.10480402680632750, -293.9171528315736737, -311.0291932777930697 ) ) ;
#60696=CARTESIAN_POINT ( 'NONE',  ( -19.44538900578974960, -288.2633913686266851, -197.8934089817844608 ) ) ;
#60698=CARTESIAN_POINT ( 'NONE',  ( 25.22466315766302358, -284.4094976428775112, -220.5068182859052968 ) ) ;
#60699=CARTESIAN_POINT ( 'NONE',  ( -112.9086949205890704, -277.5739520403763549, -284.3542396196921231 ) ) ;
#60700=CARTESIAN_POINT ( 'NONE',  ( 6.057492742986257284, -291.0301712839860215, -207.7276567024939880 ) ) ;
#60701=CARTESIAN_POINT ( 'NONE',  ( -96.33247147748181760, -286.6863907198519428, -226.1932942912849285 ) ) ;
#60702=CARTESIAN_POINT ( 'NONE',  ( -43.26616232028376174, -278.8881364826787035, -344.1369592954919199 ) ) ;
#60703=CARTESIAN_POINT ( 'NONE',  ( -18.34619209592591105, -287.7173918965106054, -196.2944349023662198 ) ) ;
#60704=CARTESIAN_POINT ( 'NONE',  ( -0.2410931236640105890, -284.5588246236179657, -335.5419864141704238 ) ) ;
#60705=CARTESIAN_POINT ( 'NONE',  ( 8.242771729229867006, -276.6146646364114758, -332.4840099729999565 ) ) ;
#60706=CARTESIAN_POINT ( 'NONE',  ( -97.05573908548733186, -277.7329307282209925, -318.9948666897630574 ) ) ;
#60707=CARTESIAN_POINT ( 'NONE',  ( -35.11783909226129197, -300.0003528430044071, -195.9203753877539782 ) ) ;
#60710=CARTESIAN_POINT ( 'NONE',  ( -36.53280109627711880, -296.2017666697079221, -194.5965636609959404 ) ) ;
#60712=CARTESIAN_POINT ( 'NONE',  ( -19.00755205941983661, -276.3173497832154339, -341.0848583818217890 ) ) ;
#60713=CARTESIAN_POINT ( 'NONE',  ( -87.78648723225141737, -274.5709710616191614, -212.6422327271353083 ) ) ;
#60714=CARTESIAN_POINT ( 'NONE',  ( 23.56795171037360603, -279.9855614980049836, -223.6188254416905465 ) ) ;
#60715=CARTESIAN_POINT ( 'NONE',  ( 18.52657235348485898, -288.6296532150673215, -221.8151588811089425 ) ) ;
#60716=CARTESIAN_POINT ( 'NONE',  ( -95.04440103841686494, -297.3915831473902358, -320.2921310073183463 ) ) ;
#60717=CARTESIAN_POINT ( 'NONE',  ( -92.40088565864948578, -297.0237916151897366, -323.6198713195057621 ) ) ;
#60718=CARTESIAN_POINT ( 'NONE',  ( -19.66315597169152696, -294.2800220465041434, -197.5923594514231354 ) ) ;
#60719=CARTESIAN_POINT ( 'NONE',  ( 23.62145660569067829, -278.9606242160397755, -226.9615563584597453 ) ) ;
#60720=CARTESIAN_POINT ( 'NONE',  ( 36.86663315238075000, -283.5562919829110911, -276.8528551379662304 ) ) ;
#60721=CARTESIAN_POINT ( 'NONE',  ( -108.0674115361805718, -294.9361323342087076, -246.9774491519044375 ) ) ;
#60722=CARTESIAN_POINT ( 'NONE',  ( -101.8521541926661769, -286.6889049307578148, -229.8044695643355624 ) ) ;
#60723=CARTESIAN_POINT ( 'NONE',  ( 34.82356774758065399, -286.6419270364220893, -283.2607376132246486 ) ) ;
#60724=CARTESIAN_POINT ( 'NONE',  ( 24.51469319637114452, -280.2928157066955919, -224.6763350482493138 ) ) ;
#60725=CARTESIAN_POINT ( 'NONE',  ( 86.36035778855256240, 82.03965494544887349, -301.7430877023235212 ) ) ;
#60727=CARTESIAN_POINT ( 'NONE',  ( -44.02208616709134503, -285.6320796258899009, -197.6461956547500733 ) ) ;
#60729=CARTESIAN_POINT ( 'NONE',  ( -110.8078930676592506, -285.3540441091186040, -292.4114867239314890 ) ) ;
#60730=CARTESIAN_POINT ( 'NONE',  ( 30.19275627893312119, -275.5117571331371664, -242.4581530986482107 ) ) ;
#60731=CARTESIAN_POINT ( 'NONE',  ( -37.77941401554981127, -290.9671244651735265, -193.6714777573613446 ) ) ;
#60732=CARTESIAN_POINT ( 'NONE',  ( 19.71346318239393725, -282.9052419346073179, -321.9950323594325141 ) ) ;
#60733=CARTESIAN_POINT ( 'NONE',  ( -112.5563778921950586, -280.2346025174884971, -257.4979923012416521 ) ) ;
#60734=CARTESIAN_POINT ( 'NONE',  ( 32.37504316569854979, -282.3048862137712831, -303.1259566819899760 ) ) ;
#60735=CARTESIAN_POINT ( 'NONE',  ( -53.28691492658257545, -283.3380690714490697, -200.3538533559491555 ) ) ;
#60736=CARTESIAN_POINT ( 'NONE',  ( -12.21535056456116841, -91.97447309684723393, -360.1559200363261084 ) ) ;
#60738=CARTESIAN_POINT ( 'NONE',  ( 21.47892920326006561, -278.1890651935221968, -316.6436477195902057 ) ) ;
#60739=CARTESIAN_POINT ( 'NONE',  ( 199.0379451319788870, 289.5412081999082829, -97.41078727901259526 ) ) ;
#60740=CARTESIAN_POINT ( 'NONE',  ( 36.76975961077297939, -279.6925852846134148, -279.6882258245543653 ) ) ;
#60741=CARTESIAN_POINT ( 'NONE',  ( -109.3748887871795574, -296.0648016639579510, -257.9067051112525633 ) ) ;
#60742=CARTESIAN_POINT ( 'NONE',  ( 32.13309633229800255, -292.6343496558510537, -237.1800675261456774 ) ) ;
#60744=CARTESIAN_POINT ( 'NONE',  ( -43.22612960531466086, -296.5540940438037865, -194.1244600998590499 ) ) ;
#60745=CARTESIAN_POINT ( 'NONE',  ( -42.74258219543229842, -287.5211522892533935, -344.0143886667376592 ) ) ;
#60746=CARTESIAN_POINT ( 'NONE',  ( 27.29864803117867211, -294.9199669210070738, -233.7529178472987041 ) ) ;
#60747=CARTESIAN_POINT ( 'NONE',  ( 28.08961680829964891, -288.4143448588559409, -236.7827668650305384 ) ) ;
#60749=CARTESIAN_POINT ( 'NONE',  ( 13.11477984448461598, -293.6786324589966739, -212.5081678321506047 ) ) ;
#60750=CARTESIAN_POINT ( 'NONE',  ( -108.7789107327551079, -284.8417871090486528, -285.7408732046596356 ) ) ;
#60751=CARTESIAN_POINT ( 'NONE',  ( -34.76056875060747586, -296.8787225071721991, -193.7587024660421662 ) ) ;
#60752=CARTESIAN_POINT ( 'NONE',  ( 23.84043921676020972, -293.7339629927249689, -223.8539382171424563 ) ) ;
#60753=CARTESIAN_POINT ( 'NONE',  ( -86.47855275024571142, -291.8833598305113810, -211.0880806614227936 ) ) ;
#60754=CARTESIAN_POINT ( 'NONE',  ( 7.981603565306609305, -288.5792021865862012, -327.5869700670832572 ) ) ;
#60757=CARTESIAN_POINT ( 'NONE',  ( -40.41427878682304708, -299.8744588190737090, -194.6073536519148206 ) ) ;
#60758=CARTESIAN_POINT ( 'NONE',  ( -36.92639498832856049, -272.8522061540618324, -193.7463297912194946 ) ) ;
#60759=CARTESIAN_POINT ( 'NONE',  ( 28.35686650998900760, -281.0493618194070677, -302.8351962049384838 ) ) ;
#60762=CARTESIAN_POINT ( 'NONE',  ( -37.13343218396168055, -276.5572309816907364, -347.3123460101353430 ) ) ;
#60763=CARTESIAN_POINT ( 'NONE',  ( -68.60311088225260789, -272.0342412623425048, -203.4954605661089033 ) ) ;
#60764=CARTESIAN_POINT ( 'NONE',  ( -77.50980347881689170, -281.3677527964491674, -207.8707562732455472 ) ) ;
#60765=CARTESIAN_POINT ( 'NONE',  ( 34.07987114704710052, -273.9554615985016994, -290.6517089689587010 ) ) ;
#60766=CARTESIAN_POINT ( 'NONE',  ( -50.03760320576009946, -299.0916068100385132, -198.0704232228478077 ) ) ;
#60767=CARTESIAN_POINT ( 'NONE',  ( -33.80710660935124423, -299.1770948104688159, -197.0513362399274229 ) ) ;
#60768=CARTESIAN_POINT ( 'NONE',  ( -98.46307687774019257, -298.7640649792687100, -224.8352926383275872 ) ) ;
#60770=CARTESIAN_POINT ( 'NONE',  ( -69.40842366796222507, -271.6524719580954184, -202.1551375255288860 ) ) ;
#60771=CARTESIAN_POINT ( 'NONE',  ( 35.81003336094614298, -294.2087214731897689, -270.7522010472350757 ) ) ;
#60772=CARTESIAN_POINT ( 'NONE',  ( 28.01813084454555636, -291.6707173162600952, -236.5459230144966227 ) ) ;
#60773=CARTESIAN_POINT ( 'NONE',  ( 82.64890176555634582, -299.5541904835127980, -195.3611179825600175 ) ) ;
#60774=CARTESIAN_POINT ( 'NONE',  ( 36.82797193290609528, -276.3014956093302317, -290.8647588486030031 ) ) ;
#60775=CARTESIAN_POINT ( 'NONE',  ( -74.27521574020947526, -273.7134378322872408, -207.3349863874383914 ) ) ;
#60777=CARTESIAN_POINT ( 'NONE',  ( 24.69751471559726852, -280.8347160513006315, -315.1542568591549411 ) ) ;
#60778=CARTESIAN_POINT ( 'NONE',  ( -25.17875651936905967, -296.8977247267555981, -344.5899816567116432 ) ) ;
#60780=CARTESIAN_POINT ( 'NONE',  ( -107.9196266375112998, -283.4947241350890863, -289.6790933721925398 ) ) ;
#60781=CARTESIAN_POINT ( 'NONE',  ( -94.88369293235605539, -281.8847434509306709, -318.7437080750573841 ) ) ;
#60782=EDGE_CURVE ( 'NONE', #47026, #6475, #30172, .T. ) ;
#60784=CARTESIAN_POINT ( 'NONE',  ( 16.95373579792595464, -274.8339509894146886, -320.0526417017233598 ) ) ;
#60785=CARTESIAN_POINT ( 'NONE',  ( 36.75636932795132594, -283.7053378330349460, -282.2790430312370518 ) ) ;
#60788=CARTESIAN_POINT ( 'NONE',  ( -76.00901147481471298, -271.9449645036021366, -204.6398238528950628 ) ) ;
#60789=CARTESIAN_POINT ( 'NONE',  ( -50.95498404725360331, -279.2258922872036919, -344.2847740383422774 ) ) ;
#60791=CARTESIAN_POINT ( 'NONE',  ( -93.31566659678372844, -285.7694239595713839, -321.1368692508020786 ) ) ;
#60793=CARTESIAN_POINT ( 'NONE',  ( -54.53526744323139042, -287.2727716132861815, -343.4164821795676517 ) ) ;
#60795=CARTESIAN_POINT ( 'NONE',  ( -106.1728823496114131, -295.6867771098327466, -244.7312974594291575 ) ) ;
#60796=CARTESIAN_POINT ( 'NONE',  ( 22.14939115793219671, -286.3046816110265240, -314.7859417202719783 ) ) ;
#60797=CARTESIAN_POINT ( 'NONE',  ( 116.7412556412048872, 151.1295779098236665, -261.7160256675778101 ) ) ;
#60798=CARTESIAN_POINT ( 'NONE',  ( -111.2423151236370273, -294.7162722502666838, -257.5665975275372261 ) ) ;
#60799=CARTESIAN_POINT ( 'NONE',  ( 21.85490609014552277, -286.6841344571441255, -318.5321637991604007 ) ) ;
#60800=CARTESIAN_POINT ( 'NONE',  ( 36.48719834334961831, -283.1285743558139529, -268.5437643391194911 ) ) ;
#60801=CARTESIAN_POINT ( 'NONE',  ( -13.75800069724405006, -280.9900435000882339, -342.5953420965402643 ) ) ;
#60802=CARTESIAN_POINT ( 'NONE',  ( -80.40750505393187098, -289.6538554281773941, -329.3675222663868567 ) ) ;
#60803=CARTESIAN_POINT ( 'NONE',  ( 33.89847087420039173, -283.2195696396389053, -288.8562226198936287 ) ) ;
#60804=CARTESIAN_POINT ( 'NONE',  ( 1.195035870662750854, -283.3264104712855556, -332.6096808700619363 ) ) ;
#60805=CARTESIAN_POINT ( 'NONE',  ( 36.11057925890029452, -289.3163342305804804, -253.4762966734355700 ) ) ;
#60806=CARTESIAN_POINT ( 'NONE',  ( -101.1933853331745183, -273.4531112965436250, -227.2696249463543552 ) ) ;
#60807=CARTESIAN_POINT ( 'NONE',  ( -31.26006513394235498, -274.1269369052573666, -193.5883830188325021 ) ) ;
#60808=CARTESIAN_POINT ( 'NONE',  ( -68.51047276076144499, -293.6204823682541587, -202.5211590025788269 ) ) ;
#60810=CARTESIAN_POINT ( 'NONE',  ( -110.4683760289727132, -281.2662352645559167, -253.7030783399848985 ) ) ;
#60811=CARTESIAN_POINT ( 'NONE',  ( -23.30680261418458343, -274.8730716088636541, -344.2587802214222279 ) ) ;
#60813=CARTESIAN_POINT ( 'NONE',  ( -112.3480179013503744, -295.1218126160890733, -256.9263604243116106 ) ) ;
#60814=CARTESIAN_POINT ( 'NONE',  ( -107.7087663347654285, -291.8585772610217077, -292.7767085358653958 ) ) ;
#60815=CARTESIAN_POINT ( 'NONE',  ( -78.90622225098150011, -272.8242154691228620, -210.1640941364211699 ) ) ;
#60816=CARTESIAN_POINT ( 'NONE',  ( -107.6690269568915994, -292.3618331913442034, -248.3009687442127529 ) ) ;
#60817=CARTESIAN_POINT ( 'NONE',  ( -49.74031641792665681, -292.8315219245278627, -198.1314937105648539 ) ) ;
#60818=CARTESIAN_POINT ( 'NONE',  ( -5.577999932653798787, -284.3887464086511159, -337.2259497909354877 ) ) ;
#60819=CARTESIAN_POINT ( 'NONE',  ( -95.22651626368973155, -292.6563028435225533, -220.4617148057882048 ) ) ;
#60820=CARTESIAN_POINT ( 'NONE',  ( -95.29836750323146077, -292.5462223569459184, -220.3978906781019873 ) ) ;
#60821=CARTESIAN_POINT ( 'NONE',  ( 32.74958095056982899, -293.6558738629894378, -290.8073247116167295 ) ) ;
#60822=CARTESIAN_POINT ( 'NONE',  ( 36.73860467801897300, -289.7037128782220066, -282.1524939225739104 ) ) ;
#60823=CARTESIAN_POINT ( 'NONE',  ( 39.61987265259269009, -281.7492517272943360, -272.7934665616442658 ) ) ;
#60824=CARTESIAN_POINT ( 'NONE',  ( -62.34504856052931387, -295.8092548418420051, -199.0579149401790460 ) ) ;
#60825=CARTESIAN_POINT ( 'NONE',  ( -76.10488502040935543, -285.3828571136864980, -203.7684064659030980 ) ) ;
#60826=CARTESIAN_POINT ( 'NONE',  ( 14.90009663019717223, -278.2916971847221248, -323.7495573974704826 ) ) ;
#60827=CARTESIAN_POINT ( 'NONE',  ( -0.6712476517365167927, -284.5390993890048321, -204.9226209660616007 ) ) ;
#60828=CARTESIAN_POINT ( 'NONE',  ( -62.02631362342228982, -275.5091540005923889, -342.0473562656083004 ) ) ;
#60829=DIRECTION ( 'NONE',  ( 0.000000000000000000, 0.000000000000000000, -1.000000000000000000 ) ) ;
#60831=CARTESIAN_POINT ( 'NONE',  ( -65.34507733012496544, -282.9359737633875511, -337.8565728542171769 ) ) ;
#60833=CARTESIAN_POINT ( 'NONE',  ( -61.93475399092118749, -280.9446255697283732, -197.7573221687828777 ) ) ;
#60834=CARTESIAN_POINT ( 'NONE',  ( 38.55475922663300281, -286.4653778678508047, -258.7605743357725601 ) ) ;
#60835=CARTESIAN_POINT ( 'NONE',  ( -23.30498707026846006, -296.6305102150933521, -343.0835497460565193 ) ) ;
#60836=CARTESIAN_POINT ( 'NONE',  ( 1.987468316123474743, -276.1694666284984692, -205.0950707262607864 ) ) ;
#60838=CARTESIAN_POINT ( 'NONE',  ( 19.65719522678299569, -276.1699848890896760, -219.2497248943195700 ) ) ;
#60839=CARTESIAN_POINT ( 'NONE',  ( -43.20920539759533341, -276.9616261248662568, -343.1249303237182744 ) ) ;
#60840=CARTESIAN_POINT ( 'NONE',  ( -110.1445828276842747, -274.7446490534849204, -253.8812187734843633 ) ) ;
#60841=CARTESIAN_POINT ( 'NONE',  ( -6.231675163225775194, -284.4616492663730014, -202.2868147826131349 ) ) ;
#60843=CARTESIAN_POINT ( 'NONE',  ( -111.7794328813565841, -291.9463672578704063, -286.6541950712156108 ) ) ;
#60844=CARTESIAN_POINT ( 'NONE',  ( 4.692086760122460731, -291.5546010140099042, -210.2373567126780358 ) ) ;
#60846=CARTESIAN_POINT ( 'NONE',  ( -22.73225063113101641, -291.9110379183019859, -198.8163664484579556 ) ) ;
#60848=CARTESIAN_POINT ( 'NONE',  ( -106.2297794422614032, -291.1959038415723171, -304.1852723105001246 ) ) ;
#60849=CARTESIAN_POINT ( 'NONE',  ( -30.26075729855522312, -280.7953690375561564, -197.5525115200956634 ) ) ;
#60851=CARTESIAN_POINT ( 'NONE',  ( -113.4662798553950438, -295.5892960423192335, -261.0583833959526032 ) ) ;
#60852=CARTESIAN_POINT ( 'NONE',  ( 27.36352340955343720, -288.7504862338125236, -312.0110527152506279 ) ) ;
#60853=CARTESIAN_POINT ( 'NONE',  ( 39.61882045983549716, -287.8644155687239277, -268.6810696876136717 ) ) ;
#60854=CARTESIAN_POINT ( 'NONE',  ( -110.3305858718521080, -284.9140566143531714, -268.1908542738848382 ) ) ;
#60855=CARTESIAN_POINT ( 'NONE',  ( -100.0921933642221262, -248.0253980568164707, -334.2282667577409825 ) ) ;
#60856=CARTESIAN_POINT ( 'NONE',  ( -114.0693070538299025, -271.3720280936893801, -283.9001697967761970 ) ) ;
#60857=CARTESIAN_POINT ( 'NONE',  ( 120.9637783430752194, 147.7793525261007517, -260.2308592555319819 ) ) ;
#60858=CARTESIAN_POINT ( 'NONE',  ( -41.87678651537783736, -276.3078880379102316, -343.3945250170900181 ) ) ;
#60859=CARTESIAN_POINT ( 'NONE',  ( -68.17991660165073142, -276.3872551470253711, -336.8822968477151107 ) ) ;
#60860=CARTESIAN_POINT ( 'NONE',  ( -111.0156482867775196, -272.5011039155673416, -247.8654095336068792 ) ) ;
#60861=CARTESIAN_POINT ( 'NONE',  ( 7.012673261725664631, -59.86950493046524002, -351.5097822906775491 ) ) ;
#60862=CARTESIAN_POINT ( 'NONE',  ( -98.41990559247783210, -276.6192401504480358, -316.4559481810226202 ) ) ;
#60864=CARTESIAN_POINT ( 'NONE',  ( -109.3384937489187365, -291.2121157218818439, -257.6443230883305091 ) ) ;
#60865=CARTESIAN_POINT ( 'NONE',  ( -51.78031750999734584, -298.6749000152849476, -194.8371281121234802 ) ) ;
#60866=CARTESIAN_POINT ( 'NONE',  ( -110.7562980512556550, -297.3359417346396754, -247.1665643613593204 ) ) ;
#60867=CARTESIAN_POINT ( 'NONE',  ( -23.51675539574290141, -295.0373054540339695, -342.0916657439329924 ) ) ;
#60869=CARTESIAN_POINT ( 'NONE',  ( -35.71747977770257876, -278.9521074997410892, -345.9165408602531784 ) ) ;
#60870=CARTESIAN_POINT ( 'NONE',  ( 39.21621148718058691, -281.1619039793872616, -278.5182402958640182 ) ) ;
#60871=CARTESIAN_POINT ( 'NONE',  ( -106.7417964493630791, -279.9462330764431499, -246.5862357033571755 ) ) ;
#60872=CARTESIAN_POINT ( 'NONE',  ( 23.56898718091759548, -277.9246538853166157, -315.7908680092711506 ) ) ;
#60873=CARTESIAN_POINT ( 'NONE',  ( -71.92599426686081188, -296.1602792394132280, -205.3906564031655364 ) ) ;
#60875=CARTESIAN_POINT ( 'NONE',  ( -95.27172446263537609, -278.0938915949686248, -314.7808465401516287 ) ) ;
#60876=CARTESIAN_POINT ( 'NONE',  ( -10.41380252585087085, -275.1974309378805970, -198.3389197026997977 ) ) ;
#60877=CARTESIAN_POINT ( 'NONE',  ( 34.60296919278211902, -286.5695158995300744, -296.5394315884936987 ) ) ;
#60878=CARTESIAN_POINT ( 'NONE',  ( -70.54101747615872853, -275.6145636479400878, -203.1093077409857983 ) ) ;
#60879=CARTESIAN_POINT ( 'NONE',  ( -6.826812122227570612, -275.2341638968416078, -340.4284423441138188 ) ) ;
#60880=CARTESIAN_POINT ( 'NONE',  ( -21.10342142747762040, -288.0355915397917101, -341.6977847904311716 ) ) ;
#60881=CARTESIAN_POINT ( 'NONE',  ( -106.5837236188485946, -284.3304859965283526, -236.9118284658580080 ) ) ;
#60882=CARTESIAN_POINT ( 'NONE',  ( -10.63069602162725147, -280.9388972310754298, -339.4407650353487611 ) ) ;
#60883=CARTESIAN_POINT ( 'NONE',  ( -6.506085041916287892, -279.0399432232309209, -203.5301494664145991 ) ) ;
#60884=CARTESIAN_POINT ( 'NONE',  ( -27.62484166460048485, -284.2563766629464794, -196.5580228042815918 ) ) ;
#60885=CARTESIAN_POINT ( 'NONE',  ( -49.03810851199094145, -291.2012050072701754, -344.4954494982267761 ) ) ;
#60886=CARTESIAN_POINT ( 'NONE',  ( -110.0171913352463093, -279.8965676159797340, -259.7413290855270702 ) ) ;
#60887=CARTESIAN_POINT ( 'NONE',  ( -92.65263417022424619, -271.2595425636271216, -219.6894121869859475 ) ) ;
#60889=CARTESIAN_POINT ( 'NONE',  ( -5.805400873493357317, -281.0442634428700899, -339.7289941723872175 ) ) ;
#60890=CARTESIAN_POINT ( 'NONE',  ( -1.635306520508392980, -296.5791324490617740, -336.3305588021367498 ) ) ;
#60891=CARTESIAN_POINT ( 'NONE',  ( -70.76836225225842725, -277.8571602945608561, -202.1215966128965249 ) ) ;
#60893=CARTESIAN_POINT ( 'NONE',  ( -105.3596130347175830, -278.8458578835282538, -297.1464907029498477 ) ) ;
#60894=CARTESIAN_POINT ( 'NONE',  ( -57.95884006883206041, -285.3178921283748650, -342.6991879834647534 ) ) ;
#60897=CARTESIAN_POINT ( 'NONE',  ( -109.0717807365721796, -292.7788345443277649, -246.4462226930556596 ) ) ;
#60899=CARTESIAN_POINT ( 'NONE',  ( 4.221867437276329404, -274.4916737333997503, -332.7908424578108111 ) ) ;
#60901=CARTESIAN_POINT ( 'NONE',  ( 26.22953056051999710, -286.1788157278412541, -227.1767770054204902 ) ) ;
#60902=CARTESIAN_POINT ( 'NONE',  ( -109.2018237356184187, -289.1720842373956089, -253.4964591964692886 ) ) ;
#60904=CARTESIAN_POINT ( 'NONE',  ( 36.09380205321358659, -274.2893168500118009, -274.3560216317447953 ) ) ;
#60905=CARTESIAN_POINT ( 'NONE',  ( -39.75249119247741447, -293.2223002679822912, -344.5698066662969268 ) ) ;
#60908=CARTESIAN_POINT ( 'NONE',  ( 35.70032196455616713, -292.3137547521488955, -292.6209623261899537 ) ) ;
#60909=CARTESIAN_POINT ( 'NONE',  ( -107.2971011534770298, -286.4630654634752318, -246.6917724943312180 ) ) ;
#60910=CARTESIAN_POINT ( 'NONE',  ( -65.09804110336834526, -287.6496057294341995, -341.1525708390706200 ) ) ;
#60911=CARTESIAN_POINT ( 'NONE',  ( 36.24454981381345675, -288.9860998229279403, -271.0234886567196213 ) ) ;
#60912=EDGE_CURVE ( 'NONE', #56563, #92061, #20246, .T. ) ;
#60914=CARTESIAN_POINT ( 'NONE',  ( 20.49138996257856249, -288.9848840174375937, -315.1913983257797440 ) ) ;
#60915=CARTESIAN_POINT ( 'NONE',  ( 29.45623181886886144, -295.9918134000988630, -305.2386621550447785 ) ) ;
#60917=CARTESIAN_POINT ( 'NONE',  ( 35.46680462655513821, -288.4541812801169840, -246.3812847724732933 ) ) ;
#60918=CARTESIAN_POINT ( 'NONE',  ( -83.99681604864225903, -275.7669178214848102, -329.8634179780800082 ) ) ;
#60919=CARTESIAN_POINT ( 'NONE',  ( -91.31118456961688423, -278.1274226897337485, -325.3269166717917074 ) ) ;
#60920=CARTESIAN_POINT ( 'NONE',  ( -31.07124718639040495, -279.7959131297903355, -193.5853962490653828 ) ) ;
#60921=CARTESIAN_POINT ( 'NONE',  ( -69.99940754903839490, -299.5996887559617221, -203.2394303311089629 ) ) ;
#60923=CARTESIAN_POINT ( 'NONE',  ( -98.18273508716090703, -283.1492142510139729, -226.4829862028017544 ) ) ;
#60925=CARTESIAN_POINT ( 'NONE',  ( -109.8074234743274076, -276.9014255598690397, -254.1913883450073683 ) ) ;
#60926=CARTESIAN_POINT ( 'NONE',  ( 35.24946140037768316, -279.7942833017772841, -289.2164599249180696 ) ) ;
#60927=CARTESIAN_POINT ( 'NONE',  ( -72.53825824055297744, -275.9893228037450967, -338.0802701167282862 ) ) ;
#60928=CARTESIAN_POINT ( 'NONE',  ( -110.7427456301928856, -298.1651816732067459, -263.2518405327273854 ) ) ;
#60929=CARTESIAN_POINT ( 'NONE',  ( 19.54494539847626911, -281.1744367786498628, -321.8722679609660418 ) ) ;
#60930=CARTESIAN_POINT ( 'NONE',  ( -71.78623215759699860, -298.5264210434215215, -205.7172929439894915 ) ) ;
#60931=CARTESIAN_POINT ( 'NONE',  ( -107.3287305190174834, -298.2656397175628058, -239.3251538602405617 ) ) ;
#60932=CARTESIAN_POINT ( 'NONE',  ( -11.47876152423410012, -274.0651263854016406, -202.0194579617432282 ) ) ;
#60933=CARTESIAN_POINT ( 'NONE',  ( 35.89748046692128014, -295.3441041799431446, -254.1456147269440748 ) ) ;
#60934=CARTESIAN_POINT ( 'NONE',  ( 32.71114548599666705, -287.3087945676935533, -238.2703115212273133 ) ) ;
#60935=CARTESIAN_POINT ( 'NONE',  ( -111.3028778141268589, -276.8298452275348041, -254.8373080206446275 ) ) ;
#60936=CARTESIAN_POINT ( 'NONE',  ( -92.81061117759203682, -291.1172771414280760, -216.8792735966704299 ) ) ;
#60937=CARTESIAN_POINT ( 'NONE',  ( 15.20664587493637754, -285.8757698668489979, -219.3505329986435299 ) ) ;
#60938=CARTESIAN_POINT ( 'NONE',  ( -112.3674735616446299, -288.5774064209878702, -268.3814107934063600 ) ) ;
#60940=CARTESIAN_POINT ( 'NONE',  ( 201.9366853066881333, 285.6703355482916322, -112.9373754057687478 ) ) ;
#60941=CARTESIAN_POINT ( 'NONE',  ( -5.771512504505313501, -288.1330864019253681, -336.2497489844104166 ) ) ;
#60943=CARTESIAN_POINT ( 'NONE',  ( -90.26721016457766211, -284.7198748291708625, -326.0371448199137490 ) ) ;
#60944=CARTESIAN_POINT ( 'NONE',  ( -22.22834588464579397, -291.2997836708109958, -195.0447033697467134 ) ) ;
#60945=CARTESIAN_POINT ( 'NONE',  ( 37.19780101539632966, -282.9515460032649230, -254.4777995071097507 ) ) ;
#60946=CARTESIAN_POINT ( 'NONE',  ( -36.77314726115923094, -281.3743265107244724, -193.8434177663166338 ) ) ;
#60947=CARTESIAN_POINT ( 'NONE',  ( -80.62784257134325117, -283.4907761331751885, -329.2058946090111817 ) ) ;
#60948=CARTESIAN_POINT ( 'NONE',  ( -93.66275172753762490, -297.2686260922384349, -217.7767815830889617 ) ) ;
#60949=CARTESIAN_POINT ( 'NONE',  ( -106.7777621129673378, -274.1854271808723524, -246.2804873080846164 ) ) ;
#60950=CARTESIAN_POINT ( 'NONE',  ( -0.4216908220641580329, -290.5655556653375129, -205.4713596146963823 ) ) ;
#60951=CARTESIAN_POINT ( 'NONE',  ( -89.51369196214632495, -272.0913581842083886, -218.7354095356930941 ) ) ;
#60954=CARTESIAN_POINT ( 'NONE',  ( -106.5437535757966998, -286.1108293599751846, -297.9310442091336313 ) ) ;
#60956=CARTESIAN_POINT ( 'NONE',  ( -5.911760247855728956, -295.7282323973454368, -340.3157560695121902 ) ) ;
#60957=CARTESIAN_POINT ( 'NONE',  ( -72.43021848497625115, -286.2261686717989733, -206.2166341382790620 ) ) ;
#60958=CARTESIAN_POINT ( 'NONE',  ( 34.97525851975475319, -274.9386665362083022, -296.2680236554453472 ) ) ;
#60959=CARTESIAN_POINT ( 'NONE',  ( -5.936167116395469456, -293.1056374952254941, -200.1542195160551785 ) ) ;
#60960=CARTESIAN_POINT ( 'NONE',  ( 9.073040986028631849, -284.8212726493908917, -210.4780879564944200 ) ) ;
#60961=CARTESIAN_POINT ( 'NONE',  ( -8.523074194401136339, -292.7524918422712972, -198.9802305487791330 ) ) ;
#60963=CARTESIAN_POINT ( 'NONE',  ( -66.33352022100316958, -289.7756429435258951, -337.4342636827961996 ) ) ;
#60964=DIRECTION ( 'NONE',  ( 1.000000000000000000, 0.000000000000000000, 0.000000000000000000 ) ) ;
#60967=CARTESIAN_POINT ( 'NONE',  ( -30.22320482856529722, -125.1503534454012936, -360.5410437172449178 ) ) ;
#60968=CARTESIAN_POINT ( 'NONE',  ( -109.3296401210003523, -286.3944112642278697, -245.0541180135221566 ) ) ;
#60969=CARTESIAN_POINT ( 'NONE',  ( -55.63300648810263738, -274.7666405000204009, -350.3538533559490702 ) ) ;
#60973=CARTESIAN_POINT ( 'NONE',  ( -36.20246041631732226, -281.9578624882905729, -343.6613786060121356 ) ) ;
#60974=CARTESIAN_POINT ( 'NONE',  ( -75.32946031783012586, -277.2110569084267127, -337.3138951266201389 ) ) ;
#60975=CARTESIAN_POINT ( 'NONE',  ( -38.40486519006801558, -282.0389554383885979, -195.5226202331257355 ) ) ;
#60976=CARTESIAN_POINT ( 'NONE',  ( -107.2154437152842945, -266.9835763933201065, -306.3795532216186643 ) ) ;
#60978=CARTESIAN_POINT ( 'NONE',  ( -31.69805762668363158, -281.5569927075723626, -346.5763551601082781 ) ) ;
#60979=CARTESIAN_POINT ( 'NONE',  ( -6.310229728316707032, -284.4819142837348522, -202.4582388971718387 ) ) ;
#60981=CARTESIAN_POINT ( 'NONE',  ( -103.1682908359319839, -274.9089003659482273, -232.7435711099594187 ) ) ;
#60982=CARTESIAN_POINT ( 'NONE',  ( -39.68473477704340269, -295.5746829940383122, -343.3975182829540245 ) ) ;
#60984=CARTESIAN_POINT ( 'NONE',  ( -9.525401424345631085, -291.1080999299807104, -202.2812549465983238 ) ) ;
#60985=CARTESIAN_POINT ( 'NONE',  ( -80.16252965506953387, -278.2664605796620663, -334.2976598376451420 ) ) ;
#60986=CARTESIAN_POINT ( 'NONE',  ( -1.722629687625949035, -274.5381631485593630, -206.6264638329723482 ) ) ;
#60987=CARTESIAN_POINT ( 'NONE',  ( 32.73173550489364914, -274.8718496277727468, -301.5252981818229614 ) ) ;
#60989=CARTESIAN_POINT ( 'NONE',  ( -44.50459460446958104, -271.9614922888616775, -195.6525544874369587 ) ) ;
#60991=CARTESIAN_POINT ( 'NONE',  ( -4.737354725767092489, -296.0563668209754837, -339.4809271487356455 ) ) ;
#60996=CARTESIAN_POINT ( 'NONE',  ( -73.93923254637256548, -284.6298300622254942, -333.9394035806447505 ) ) ;
#60997=CARTESIAN_POINT ( 'NONE',  ( 32.64152977366871511, -283.6955925247962114, -300.0983151194007519 ) ) ;
#60998=CARTESIAN_POINT ( 'NONE',  ( -92.64166952185115633, -283.2203034464520783, -318.1902739854505739 ) ) ;
#60999=CARTESIAN_POINT ( 'NONE',  ( 32.85288048449277909, -274.2510478427392968, -293.1462286413533889 ) ) ;
#61000=CARTESIAN_POINT ( 'NONE',  ( -33.40746527298313140, -284.8625506324412981, -344.5047825522538574 ) ) ;
#61001=CARTESIAN_POINT ( 'NONE',  ( -40.55519323025595924, -275.5731334400442734, -343.9969387944634036 ) ) ;
#61002=CARTESIAN_POINT ( 'NONE',  ( -5.184822844517078089, -275.5653237701049534, -204.4673361643625924 ) ) ;
#61004=CARTESIAN_POINT ( 'NONE',  ( -53.73601682802289048, -280.6498880562636487, -195.2374593115058303 ) ) ;
#61008=CARTESIAN_POINT ( 'NONE',  ( -26.81651820911489281, -288.0449209414952065, -195.2783111190236127 ) ) ;
#61009=CARTESIAN_POINT ( 'NONE',  ( -12.96405449157867729, -293.9243993690338925, -339.3951554032333320 ) ) ;
#61010=CARTESIAN_POINT ( 'NONE',  ( -113.9045171092163855, -289.9974451713500230, -262.6389360753772166 ) ) ;
#61011=CARTESIAN_POINT ( 'NONE',  ( 15.77208358223047568, -285.0570126895580643, -218.8159921888677957 ) ) ;
#61012=CARTESIAN_POINT ( 'NONE',  ( 35.86238062741225718, -286.0284778067418188, -262.8419772613049759 ) ) ;
#61013=CARTESIAN_POINT ( 'NONE',  ( -86.58677046857999926, -289.5969896313118852, -215.0391265426446807 ) ) ;
#61014=CARTESIAN_POINT ( 'NONE',  ( -5.640974070528423923, -287.6836297779189522, -204.1491145502959341 ) ) ;
#61015=CARTESIAN_POINT ( 'NONE',  ( -112.3763323641495617, -276.5726598156686009, -268.7510845046080590 ) ) ;
#61016=CARTESIAN_POINT ( 'NONE',  ( 16.11010880861870476, -286.7095308492217214, -324.7423389381839911 ) ) ;
#61017=CARTESIAN_POINT ( 'NONE',  ( 21.40888422927025658, -288.9115637186320100, -223.7212466847239227 ) ) ;
#61018=CARTESIAN_POINT ( 'NONE',  ( 22.66293520227894476, -286.1695701959802136, -315.6322143759053915 ) ) ;
#61019=CARTESIAN_POINT ( 'NONE',  ( -48.35226777259792641, -284.1369962038935455, -342.7639898024030458 ) ) ;
#61020=CARTESIAN_POINT ( 'NONE',  ( -68.57179437363420504, -291.4617104075195471, -338.7470438510124495 ) ) ;
#61023=CARTESIAN_POINT ( 'NONE',  ( -98.76549261286159265, -299.0665086796157652, -226.3562101160223392 ) ) ;
#61024=CARTESIAN_POINT ( 'NONE',  ( 28.21915272646883821, -279.0672813084037784, -233.9361921875835151 ) ) ;
#61025=CARTESIAN_POINT ( 'NONE',  ( -56.13936762918189771, -291.0132844020712923, -195.8025523022004677 ) ) ;
#61026=CARTESIAN_POINT ( 'NONE',  ( -82.41680434362213248, -295.8252478169389974, -211.8611398112899167 ) ) ;
#61027=CARTESIAN_POINT ( 'NONE',  ( 33.79666536730879756, -280.4795664751766253, -288.8659133817051270 ) ) ;
#61028=CARTESIAN_POINT ( 'NONE',  ( -70.10310767812671884, -271.6969289599835520, -203.5179853726775150 ) ) ;
#61029=CARTESIAN_POINT ( 'NONE',  ( -31.54687434219142972, -296.2927845427873876, -343.6759092583322968 ) ) ;
#61031=CARTESIAN_POINT ( 'NONE',  ( -83.21176718700370145, -272.0127664526270905, -209.1839981144141518 ) ) ;
#61032=CARTESIAN_POINT ( 'NONE',  ( 3.661382102867504873, -292.7488736743098912, -334.3974372014749861 ) ) ;
#61033=AXIS2_PLACEMENT_3D ( 'NONE', #55663, #12574, #76027 ) ;
#61034=CARTESIAN_POINT ( 'NONE',  ( -47.09034410794024694, -293.3511698088163371, -197.4204650049438499 ) ) ;
#61036=CARTESIAN_POINT ( 'NONE',  ( 20.30381946967143136, -293.7211270258691229, -225.2898041768781354 ) ) ;
#61037=DIRECTION ( 'NONE',  ( -1.000000000000000000, -0.000000000000000000, -0.000000000000000000 ) ) ;
#61039=CARTESIAN_POINT ( 'NONE',  ( -82.90908606689013993, -281.6916673415432228, -330.4435144732991603 ) ) ;
#61040=CARTESIAN_POINT ( 'NONE',  ( -28.89597898657987329, -294.9422432129071012, -342.9219226700741388 ) ) ;
#61042=CARTESIAN_POINT ( 'NONE',  ( -27.37210054310012097, -282.9289394269802074, -346.7663427963810250 ) ) ;
#61043=CARTESIAN_POINT ( 'NONE',  ( 37.36711674329588817, -283.3238512005738130, -258.7128930921769552 ) ) ;
#61044=CARTESIAN_POINT ( 'NONE',  ( -57.74624281317331764, -285.4625034913224795, -196.0804570033125174 ) ) ;
#61045=CARTESIAN_POINT ( 'NONE',  ( -112.0749672451352694, -288.6133317056160195, -265.5940688975930470 ) ) ;
#61046=CARTESIAN_POINT ( 'NONE',  ( -21.88550880992767844, -281.3374224339623311, -345.0860395338518174 ) ) ;
#61048=EDGE_CURVE ( 'NONE', #11917, #54554, #63902, .T. ) ;
#61049=CARTESIAN_POINT ( 'NONE',  ( -34.69132753772392164, -287.9399116452678982, -347.0061963352706584 ) ) ;
#61051=CARTESIAN_POINT ( 'NONE',  ( -8.903984791742105998, -296.2740060686122661, -338.4758055268594035 ) ) ;
#61052=CARTESIAN_POINT ( 'NONE',  ( -68.75641037366860076, -278.8823140277010566, -340.0297160302223460 ) ) ;
#61053=CARTESIAN_POINT ( 'NONE',  ( 36.73559792748903874, -291.7497481715136018, -284.2495702668428521 ) ) ;
#61054=CARTESIAN_POINT ( 'NONE',  ( -108.6264690372655650, -278.4283129252535218, -254.4745154352592351 ) ) ;
#61055=CARTESIAN_POINT ( 'NONE',  ( 19.41422694405919103, -293.0108840301961095, -218.3249310863966457 ) ) ;
#61057=CARTESIAN_POINT ( 'NONE',  ( -60.05334970038846620, -283.8400460926261530, -198.2406793992194025 ) ) ;
#61058=CARTESIAN_POINT ( 'NONE',  ( -76.74197839477417915, -279.5793236921047651, -334.2385306546398738 ) ) ;
#61059=CARTESIAN_POINT ( 'NONE',  ( 29.70065859092902727, -293.0061559313315911, -299.8353539322247343 ) ) ;
#61060=CARTESIAN_POINT ( 'NONE',  ( -91.82532259941586972, -271.2771939937046000, -218.5585286426650384 ) ) ;
#61064=CARTESIAN_POINT ( 'NONE',  ( 34.12646259419165062, -293.2606131899670459, -285.5964177754868274 ) ) ;
#61065=DIRECTION ( 'NONE',  ( 0.000000000000000000, 0.000000000000000000, 1.000000000000000000 ) ) ;
#61066=CARTESIAN_POINT ( 'NONE',  ( -37.37352853689063181, -286.5523547857346784, -340.3611179825599606 ) ) ;
#61067=CARTESIAN_POINT ( 'NONE',  ( -80.48285289593823677, -296.5420516916870497, -206.8018494937207095 ) ) ;
#61068=CARTESIAN_POINT ( 'NONE',  ( -43.64246329926915280, -287.2894238705015937, -194.0612411544955478 ) ) ;
#61069=CARTESIAN_POINT ( 'NONE',  ( -78.17617355877236207, -289.4512879364974651, -330.9326818215802746 ) ) ;
#61070=CARTESIAN_POINT ( 'NONE',  ( -93.24003146035299494, -279.3949705593958583, -318.3828246173822549 ) ) ;
#61071=CARTESIAN_POINT ( 'NONE',  ( -102.1120315737294106, -298.7950788001650153, -234.5452252006443814 ) ) ;
#61073=CARTESIAN_POINT ( 'NONE',  ( 9.541903779084519144, -279.5083501258902174, -213.8231064393754366 ) ) ;
#61075=CARTESIAN_POINT ( 'NONE',  ( -20.51140391415574271, -297.9241948780934877, -193.3831815583004641 ) ) ;
#61076=CARTESIAN_POINT ( 'NONE',  ( -110.1235490894070921, -292.6744282285387726, -254.7368847777409826 ) ) ;
#61077=CARTESIAN_POINT ( 'NONE',  ( 35.51604006505954914, -294.8690642353187741, -248.0409452780923232 ) ) ;
#61079=CARTESIAN_POINT ( 'NONE',  ( -110.0751374380402012, -291.3001388190311900, -263.0303768795393466 ) ) ;
#61081=CARTESIAN_POINT ( 'NONE',  ( 18.52120524151442282, -290.9841152761231342, -219.1786865759690102 ) ) ;
#61082=CARTESIAN_POINT ( 'NONE',  ( -108.8705253541002378, -297.2480267019304847, -241.7683982936289340 ) ) ;
#61084=CARTESIAN_POINT ( 'NONE',  ( -92.75768271131310883, -296.8957873112638595, -222.7902687756990474 ) ) ;
#61087=CARTESIAN_POINT ( 'NONE',  ( -104.5361973912015401, -291.6004754151089742, -306.5219709673091870 ) ) ;
#61088=CARTESIAN_POINT ( 'NONE',  ( -88.52914483777347243, -293.9090924074131408, -206.2264541496106460 ) ) ;
#61090=CARTESIAN_POINT ( 'NONE',  ( -40.06553033087357818, -288.0179972217203499, -195.5773685568224494 ) ) ;
#61092=CARTESIAN_POINT ( 'NONE',  ( 35.92131433049313216, -273.3549442841310793, -255.0485703507428070 ) ) ;
#61093=CARTESIAN_POINT ( 'NONE',  ( 20.31210428493328735, -278.1262986156413035, -317.4699913169359320 ) ) ;
#61094=CARTESIAN_POINT ( 'NONE',  ( -25.14962116923609159, -290.2885025539889057, -196.8738378625922110 ) ) ;
#61095=CARTESIAN_POINT ( 'NONE',  ( -68.48562749862624344, -279.3173872864225586, -339.4430911085285061 ) ) ;
#61097=CARTESIAN_POINT ( 'NONE',  ( -70.26825741715420293, -282.8465380153288606, -335.6417582431500932 ) ) ;
#61098=CARTESIAN_POINT ( 'NONE',  ( -114.0753947170813660, -279.6160508904845301, -271.6171115694641571 ) ) ;
#61099=CARTESIAN_POINT ( 'NONE',  ( 33.96048603263501064, -279.9886430435101374, -242.2161422086392122 ) ) ;
#61100=CARTESIAN_POINT ( 'NONE',  ( 43.74668670635536216, 12.16893915163007733, -329.0196699399712088 ) ) ;
#61101=CARTESIAN_POINT ( 'NONE',  ( 39.47207304594562061, -276.5033894309517564, -271.1572026706411407 ) ) ;
#61103=CARTESIAN_POINT ( 'NONE',  ( -0.3982295024258034610, -276.0541650090034977, -203.5788463470345562 ) ) ;
#61104=CARTESIAN_POINT ( 'NONE',  ( -102.0455923789670294, -275.4805209788415823, -239.2376011013261916 ) ) ;
#61109=CARTESIAN_POINT ( 'NONE',  ( -56.13160983291376738, -290.3794706047376053, -341.2740767488010079 ) ) ;
#61110=CARTESIAN_POINT ( 'NONE',  ( -102.9125124544062260, -291.8046479014522561, -308.8636117106902361 ) ) ;
#61111=CARTESIAN_POINT ( 'NONE',  ( -110.4695548327274253, -289.9258994683572155, -268.4508303017759658 ) ) ;
#61112=CARTESIAN_POINT ( 'NONE',  ( -85.46953200798462547, -284.9144249481172437, -210.3341348700142817 ) ) ;
#61114=CARTESIAN_POINT ( 'NONE',  ( 31.06856185501822765, -280.3187569898180982, -298.0464294114511858 ) ) ;
#61115=CARTESIAN_POINT ( 'NONE',  ( -7.703931367187408341, -290.5200834829938685, -338.4783187292500770 ) ) ;
#61116=CARTESIAN_POINT ( 'NONE',  ( -94.83800723505883923, -282.3865700833115966, -316.4776460841226822 ) ) ;
#61117=CARTESIAN_POINT ( 'NONE',  ( 35.51944217815985638, -282.7363620315924777, -260.3658404532135933 ) ) ;
#61118=CARTESIAN_POINT ( 'NONE',  ( 36.16356842236982061, -288.7725403371177322, -292.5381252622189550 ) ) ;
#61120=CARTESIAN_POINT ( 'NONE',  ( -108.6682003086464761, -279.2538075289531889, -254.4760374648383845 ) ) ;
#61121=CARTESIAN_POINT ( 'NONE',  ( -92.51538155098648986, -290.0790488923523753, -217.1455390022598522 ) ) ;
#61122=CARTESIAN_POINT ( 'NONE',  ( -110.5286180618309402, -285.0596027625623492, -293.8103408665072038 ) ) ;
#61123=CARTESIAN_POINT ( 'NONE',  ( -12.72933335143210343, -286.8560923676025709, -197.4655879084660626 ) ) ;
#61124=CARTESIAN_POINT ( 'NONE',  ( -82.79306352419723680, -283.8600878613000305, -327.5501751696892825 ) ) ;
#61127=CARTESIAN_POINT ( 'NONE',  ( -58.61493065692390303, -293.6403389697273383, -197.6441657562770615 ) ) ;
#61129=CARTESIAN_POINT ( 'NONE',  ( 32.87844883609535174, -291.8474731359370935, -239.9896025288758779 ) ) ;
#61131=CARTESIAN_POINT ( 'NONE',  ( 32.73806904357483916, -274.8920971404298825, -291.6703697371067960 ) ) ;
#61132=CARTESIAN_POINT ( 'NONE',  ( -110.7050425453647335, -295.6102657435727679, -293.4515254851738746 ) ) ;
#61133=CARTESIAN_POINT ( 'NONE',  ( -9.447257154994359141, -290.9031850680901812, -202.0967877339206780 ) ) ;
#61134=CARTESIAN_POINT ( 'NONE',  ( 20.47143900786562654, -292.4361053614398429, -316.5940276273177005 ) ) ;
#61135=CARTESIAN_POINT ( 'NONE',  ( -22.67620711218559748, -293.4491472572595967, -198.4441254269270303 ) ) ;
#61138=CARTESIAN_POINT ( 'NONE',  ( 27.89738819161332017, -291.0551154101930251, -233.0262846567994188 ) ) ;
#61139=CARTESIAN_POINT ( 'NONE',  ( 22.72937136620262777, -296.1659469225631938, -315.2873301167448403 ) ) ;
#61140=CARTESIAN_POINT ( 'NONE',  ( 30.70824988230531716, -288.8560226751339428, -297.5647694007143969 ) ) ;
#61141=CARTESIAN_POINT ( 'NONE',  ( -38.49397032642803396, -279.0464212675569229, -345.7075119251946944 ) ) ;
#61142=CARTESIAN_POINT ( 'NONE',  ( -82.32556824998403044, -276.4460758600843064, -332.3648301806337031 ) ) ;
#61144=CARTESIAN_POINT ( 'NONE',  ( -26.22845828252329525, -297.3851421146307530, -193.5240625362837363 ) ) ;
#61145=CARTESIAN_POINT ( 'NONE',  ( -11.21528089560723274, -278.4749786837091960, -200.6020470126230464 ) ) ;
#61146=CARTESIAN_POINT ( 'NONE',  ( -111.0587526299876515, -276.7074067776957804, -289.7058756206711791 ) ) ;
#61147=CARTESIAN_POINT ( 'NONE',  ( -107.1701259474203596, -295.5410148275258848, -247.2819022478191471 ) ) ;
#61148=CARTESIAN_POINT ( 'NONE',  ( -109.1683679093899144, -274.8324875907955516, -248.5990953173099456 ) ) ;
#61149=CARTESIAN_POINT ( 'NONE',  ( -65.86055204674019592, -274.3203211373043473, -203.0516256829406814 ) ) ;
#61151=CARTESIAN_POINT ( 'NONE',  ( -67.42099764189555344, -287.4648311380520909, -339.4526707679829087 ) ) ;
#61152=CARTESIAN_POINT ( 'NONE',  ( 33.50969327064054681, -275.1534774108990860, -252.7804451287752272 ) ) ;
#61153=CARTESIAN_POINT ( 'NONE',  ( 38.55686124440615004, -287.3888839710847947, -257.3063253781451749 ) ) ;
#61154=CARTESIAN_POINT ( 'NONE',  ( 17.85844122611258911, -300.7197990699097545, -194.9873902654363746 ) ) ;
#61155=CARTESIAN_POINT ( 'NONE',  ( -97.08293841898321830, -293.9342288339367997, -315.4489961794517967 ) ) ;
#61156=CARTESIAN_POINT ( 'NONE',  ( -104.2813765694811536, -283.2575490106374332, -308.1947425455101666 ) ) ;
#61158=CARTESIAN_POINT ( 'NONE',  ( -2.901071364674446595, -278.5071072935193683, -203.7222381759013956 ) ) ;
#61160=CARTESIAN_POINT ( 'NONE',  ( -110.7039167626998193, -289.3004684929671839, -273.9129526877747480 ) ) ;
#61162=CARTESIAN_POINT ( 'NONE',  ( -38.91467087911562572, -290.0322565414983274, -195.3776103601423699 ) ) ;
#61163=CARTESIAN_POINT ( 'NONE',  ( -1.401246139056952167, -276.0580396519193869, -206.0116758496154716 ) ) ;
#61164=CARTESIAN_POINT ( 'NONE',  ( 33.03041228520542205, -283.3607774926060756, -300.2683200310597726 ) ) ;
#61166=CARTESIAN_POINT ( 'NONE',  ( -112.9017001288127773, -270.6323071252278396, -270.3367248692900375 ) ) ;
#61167=CARTESIAN_POINT ( 'NONE',  ( -29.44465309213074988, -282.9494795944524412, -342.9832183258961891 ) ) ;
#61168=CARTESIAN_POINT ( 'NONE',  ( -40.82082042459323645, -275.4329483492452368, -196.8040741209401574 ) ) ;
#61169=CARTESIAN_POINT ( 'NONE',  ( 35.74770136578801782, -276.2991583901867898, -266.1194408566408356 ) ) ;
#61170=CARTESIAN_POINT ( 'NONE',  ( 30.59192902350789467, -283.9714973125862798, -302.2644155037862106 ) ) ;
#61172=CARTESIAN_POINT ( 'NONE',  ( 203.2340568605973772, 295.9509986211770638, -54.00000000006198064 ) ) ;
#61173=CARTESIAN_POINT ( 'NONE',  ( -30.59306562501696902, -294.8023632282826725, -347.0648071822886322 ) ) ;
#61174=CARTESIAN_POINT ( 'NONE',  ( -94.53116604107296439, -287.1982117339554748, -222.3901705825836927 ) ) ;
#61176=CARTESIAN_POINT ( 'NONE',  ( -117.3452863284742733, -275.1604526064901393, -261.3791111993605227 ) ) ;
#61177=CARTESIAN_POINT ( 'NONE',  ( -96.03248285041129861, -277.0795735837839970, -319.9752884853033947 ) ) ;
#61178=CARTESIAN_POINT ( 'NONE',  ( -88.96463199667282140, -288.1633067178807437, -326.4103224293067456 ) ) ;
#61179=CARTESIAN_POINT ( 'NONE',  ( -52.24791192551646901, -287.3779483856088746, -198.1910923459612661 ) ) ;
#61180=CARTESIAN_POINT ( 'NONE',  ( -89.78827780428588312, -279.5644231429540127, -322.6577223796755902 ) ) ;
#61181=CARTESIAN_POINT ( 'NONE',  ( -21.12683496526869575, -287.6815331340808939, -195.6906121650895614 ) ) ;
#61182=CARTESIAN_POINT ( 'NONE',  ( 31.85726556961443379, -283.1746699740484701, -241.4387426918657980 ) ) ;
#61183=CARTESIAN_POINT ( 'NONE',  ( 39.70741351921355999, -275.7289421212855700, -271.1695245178572691 ) ) ;
#61184=CARTESIAN_POINT ( 'NONE',  ( -112.7940561520883591, -278.1925549419570984, -285.7866900977512614 ) ) ;
#61185=CARTESIAN_POINT ( 'NONE',  ( -111.6784197933859275, -298.4216015120937300, -274.2811058297753561 ) ) ;
#61189=CARTESIAN_POINT ( 'NONE',  ( -112.3417001280813849, -275.0519495502701943, -270.3929463913696054 ) ) ;
#61190=CARTESIAN_POINT ( 'NONE',  ( 96.48985628060853514, -297.8500639586717966, -194.6381542544558840 ) ) ;
#61192=CARTESIAN_POINT ( 'NONE',  ( -83.05013735437303524, -277.2047449216918267, -327.4238423791767900 ) ) ;
#61193=CARTESIAN_POINT ( 'NONE',  ( -93.86271078175940374, -274.4642613820264501, -218.6369681025128955 ) ) ;
#61194=CARTESIAN_POINT ( 'NONE',  ( 36.76103030286353857, -280.3586051216105943, -250.2711410957494422 ) ) ;
#61195=CARTESIAN_POINT ( 'NONE',  ( 34.69142250384854265, -289.0903158901492702, -253.3004363684986799 ) ) ;
#61196=CARTESIAN_POINT ( 'NONE',  ( -112.9628185808622192, -297.9386015700267194, -280.9529787642888436 ) ) ;
#61197=CARTESIAN_POINT ( 'NONE',  ( -53.19202163374237813, -296.4559739928315025, -345.3605309012414182 ) ) ;
#61199=CARTESIAN_POINT ( 'NONE',  ( 7.761443472523162690, -294.6698512498923037, -210.6473435179227067 ) ) ;
#61200=CARTESIAN_POINT ( 'NONE',  ( -65.48249506226881067, -277.6832125685359642, -201.0204799113909928 ) ) ;
#61201=CARTESIAN_POINT ( 'NONE',  ( 16.28001923175133570, -282.7404475058839921, -218.6539394991268921 ) ) ;
#61202=CARTESIAN_POINT ( 'NONE',  ( -50.17867404431141409, -295.9668801133246916, -197.0363179762350114 ) ) ;
#61203=CARTESIAN_POINT ( 'NONE',  ( -73.87433644447233405, -285.1287193937960183, -337.2915549751027129 ) ) ;
#61205=CARTESIAN_POINT ( 'NONE',  ( 22.25085615772718839, -285.8772262047522190, -227.5794554563788381 ) ) ;
#61206=CARTESIAN_POINT ( 'NONE',  ( 162.8811038778437421, 219.0089487911489812, -204.8009164393295123 ) ) ;
#61208=CARTESIAN_POINT ( 'NONE',  ( 29.98291127326664451, -286.8380113863557312, -241.9550033858817528 ) ) ;
#61210=CARTESIAN_POINT ( 'NONE',  ( -69.04606380591251025, -284.5390704959723394, -340.2061668788211364 ) ) ;
#61211=CARTESIAN_POINT ( 'NONE',  ( 19.01246479769613273, -275.2275219379220630, -223.9251881180274495 ) ) ;
#61212=CARTESIAN_POINT ( 'NONE',  ( -30.90186084065257788, -284.9267281581383600, -194.0161342613318425 ) ) ;
#61213=CARTESIAN_POINT ( 'NONE',  ( -69.48102541539080335, -290.5593684631805331, -200.7152596714730635 ) ) ;
#61214=CARTESIAN_POINT ( 'NONE',  ( 1.245296188414876104, -281.4951930970142939, -203.9389880269300477 ) ) ;
#61216=CARTESIAN_POINT ( 'NONE',  ( -102.8266319910048452, -280.5888348872528013, -231.0865159685884578 ) ) ;
#61217=CARTESIAN_POINT ( 'NONE',  ( 38.12565972344505383, -282.0753262874368943, -285.5407717551344149 ) ) ;
#61218=CARTESIAN_POINT ( 'NONE',  ( 7.450504543161054372, -284.1952119285919025, -214.2458315076590907 ) ) ;
#61219=CARTESIAN_POINT ( 'NONE',  ( -107.3199604355249051, -262.9330320181824732, -317.7331714456881286 ) ) ;
#61221=CARTESIAN_POINT ( 'NONE',  ( 35.91084419087310664, -277.3546180294409282, -254.9985571154810771 ) ) ;
#61222=CARTESIAN_POINT ( 'NONE',  ( -104.9347473080156163, -255.2955550898405193, -326.2820073762666766 ) ) ;
#61223=CARTESIAN_POINT ( 'NONE',  ( 34.90934673734872007, -279.8149557726275702, -289.1638438378815863 ) ) ;
#61224=CARTESIAN_POINT ( 'NONE',  ( -32.06026631913207581, -296.7465544766477024, -346.1771035322989860 ) ) ;
#61225=CARTESIAN_POINT ( 'NONE',  ( -94.02684526694497436, -295.2480743567660966, -316.5401590733378612 ) ) ;
#61226=CARTESIAN_POINT ( 'NONE',  ( -96.52750866996859713, -290.7215602056205626, -221.1821706045000155 ) ) ;
#61228=CARTESIAN_POINT ( 'NONE',  ( -113.3588826612229639, -295.0292658904818950, -278.1067136155596700 ) ) ;
#61229=CARTESIAN_POINT ( 'NONE',  ( 29.54350030742865485, -285.5354398154176465, -239.1712097474611767 ) ) ;
#61230=CARTESIAN_POINT ( 'NONE',  ( 33.53302600010901813, -295.7003214018989752, -292.4436603379149915 ) ) ;
#61231=CARTESIAN_POINT ( 'NONE',  ( -9.320762240904400642, -287.7414342166643451, -202.4058504348868723 ) ) ;
#61233=CARTESIAN_POINT ( 'NONE',  ( 39.20553797929906636, -294.4209674763781663, -264.5869902942046679 ) ) ;
#61234=CARTESIAN_POINT ( 'NONE',  ( -97.57953334127418543, -284.4683925823658797, -311.7940750023726650 ) ) ;
#61235=CARTESIAN_POINT ( 'NONE',  ( -112.4961179033775522, -295.5343145222853423, -255.4673260894332429 ) ) ;
#61236=CARTESIAN_POINT ( 'NONE',  ( -103.0829987075748448, -291.8763781031692588, -230.4811240711913456 ) ) ;
#61237=CARTESIAN_POINT ( 'NONE',  ( -101.6359888281575365, -291.6015297351016216, -228.0071148928085165 ) ) ;
#61238=CARTESIAN_POINT ( 'NONE',  ( -108.3499231793004327, -290.4953967718241756, -287.2972410231224671 ) ) ;
#61240=CARTESIAN_POINT ( 'NONE',  ( 82.64890176555634582, -299.5541904835127980, -197.7570935515975918 ) ) ;
#61241=CARTESIAN_POINT ( 'NONE',  ( -36.92950625991289115, -299.9176694314135716, -194.5961815503768548 ) ) ;
#61242=CARTESIAN_POINT ( 'NONE',  ( -113.1490700837806003, -271.4900487068189250, -258.9884009044006348 ) ) ;
#61243=CARTESIAN_POINT ( 'NONE',  ( 33.99229161686636758, -280.3928902655889033, -253.7819120100527357 ) ) ;
#61245=CARTESIAN_POINT ( 'NONE',  ( 39.56951231019630200, -275.0341785101417145, -268.3136062407267559 ) ) ;
#61246=CARTESIAN_POINT ( 'NONE',  ( -109.8275895882569131, -294.8575033894813373, -283.7165863621206654 ) ) ;
#61247=CARTESIAN_POINT ( 'NONE',  ( -54.21199183059562188, -279.1313864684050259, -342.7070051932167871 ) ) ;
#61248=CARTESIAN_POINT ( 'NONE',  ( 35.59139518428406745, -273.5121605587906970, -256.5181020326321004 ) ) ;
#61249=CARTESIAN_POINT ( 'NONE',  ( -110.1320633464270173, -297.8858419255379317, -260.5588414901434362 ) ) ;
#61250=CARTESIAN_POINT ( 'NONE',  ( -66.95676868256512648, -298.7343323176042418, -203.2864081614265217 ) ) ;
#61251=CARTESIAN_POINT ( 'NONE',  ( -72.92537711763402797, -299.1892153442483959, -202.9215531611147298 ) ) ;
#61252=CARTESIAN_POINT ( 'NONE',  ( -46.65223985163488862, -271.9546172902489047, -195.5833094340492551 ) ) ;
#61253=CARTESIAN_POINT ( 'NONE',  ( 35.00743672500120596, -294.0657235268195109, -259.8971290277253843 ) ) ;
#61254=CARTESIAN_POINT ( 'NONE',  ( -0.9496202824729688130, -291.1200860321305868, -206.3856654188712412 ) ) ;
#61257=CARTESIAN_POINT ( 'NONE',  ( 33.65433975390517674, -275.6655776260096786, -240.5741054012914333 ) ) ;
#61258=CARTESIAN_POINT ( 'NONE',  ( -37.15381829456106999, -298.3878581469235769, -197.3371132438529685 ) ) ;
#61259=CARTESIAN_POINT ( 'NONE',  ( 37.99514284250686558, -283.4904078664116014, -267.1028007542923888 ) ) ;
#61260=CARTESIAN_POINT ( 'NONE',  ( -67.70116118732174471, -282.1271301440829689, -340.5864794834035933 ) ) ;
#61262=CARTESIAN_POINT ( 'NONE',  ( -73.88629885156321109, -282.7476298618543638, -333.7994023444343838 ) ) ;
#61264=CARTESIAN_POINT ( 'NONE',  ( -82.79533508452522028, -281.6714023077923343, -330.2929990674005012 ) ) ;
#61265=CARTESIAN_POINT ( 'NONE',  ( 34.73807216750496707, -274.3209220712727756, -285.1895145423513327 ) ) ;
#61266=CARTESIAN_POINT ( 'NONE',  ( -34.79805432837309809, -282.0841675863708247, -195.3541177916236222 ) ) ;
#61269=CARTESIAN_POINT ( 'NONE',  ( -83.08342137367077385, -271.8379385012563034, -209.3513851557187309 ) ) ;
#61270=CARTESIAN_POINT ( 'NONE',  ( -100.5413933777107900, -280.0042594206789772, -311.1479043380187477 ) ) ;
#61272=CARTESIAN_POINT ( 'NONE',  ( -92.87827025563065320, -287.1838003544532398, -219.0496198482255181 ) ) ;
#61275=CARTESIAN_POINT ( 'NONE',  ( 23.62112409745348174, -286.1473191155689619, -314.1341037901555637 ) ) ;
#61278=CARTESIAN_POINT ( 'NONE',  ( -108.8605086271576994, -295.5635368191865950, -253.8629199863998167 ) ) ;
#61279=CARTESIAN_POINT ( 'NONE',  ( -26.31441578364136902, -287.0500409453898669, -343.8246395955183061 ) ) ;
#61281=CARTESIAN_POINT ( 'NONE',  ( -103.2363275121843742, -294.0761666386493971, -306.1786936673113928 ) ) ;
#61282=CARTESIAN_POINT ( 'NONE',  ( -7.595381012763462891, -284.9148164410742083, -200.0350266332745264 ) ) ;
#61283=CARTESIAN_POINT ( 'NONE',  ( 18.55729277409077937, -282.4732417805408318, -222.1572573345381159 ) ) ;
#61284=CARTESIAN_POINT ( 'NONE',  ( -91.72436864482629915, -282.0543659227286639, -323.4318196740168787 ) ) ;
#61285=CARTESIAN_POINT ( 'NONE',  ( -3.366371430787300500, -288.5907394986638224, -335.0288430176313454 ) ) ;
#61286=CARTESIAN_POINT ( 'NONE',  ( -74.82139689060470289, -280.9683005205362178, -206.9728690477283521 ) ) ;
#61287=CARTESIAN_POINT ( 'NONE',  ( -41.06961524653080176, -280.8068708255669890, -197.2946798859501030 ) ) ;
#61288=CARTESIAN_POINT ( 'NONE',  ( 17.14440229512996794, -288.8039296238887346, -218.2313875354229822 ) ) ;
#61289=CARTESIAN_POINT ( 'NONE',  ( -87.46387014799482529, -297.5422283037543139, -211.8377003311239832 ) ) ;
#61291=CARTESIAN_POINT ( 'NONE',  ( -66.22722039019882345, -273.6843462982731694, -198.9702939169441436 ) ) ;
#61292=CARTESIAN_POINT ( 'NONE',  ( -11.71876487408031942, -294.3671831855201049, -200.1967479695250915 ) ) ;
#61294=CARTESIAN_POINT ( 'NONE',  ( 10.64812456238590066, -278.9090924074130839, -330.4860931364851808 ) ) ;
#61296=CARTESIAN_POINT ( 'NONE',  ( 9.366427474328158809, -274.4122399590690975, -329.3205112761508531 ) ) ;
#61298=CARTESIAN_POINT ( 'NONE',  ( -40.38765757333001716, -296.4144736929819146, -194.1704320683369360 ) ) ;
#61299=CARTESIAN_POINT ( 'NONE',  ( -5.255838620602536260, -273.8345196278169169, -204.6632560731589479 ) ) ;
#61300=CARTESIAN_POINT ( 'NONE',  ( -100.3140262802480578, -292.5944743208195291, -232.0832668081976919 ) ) ;
#61301=CARTESIAN_POINT ( 'NONE',  ( -0.7315389881543790107, -284.3188441072293244, -334.6858419652319299 ) ) ;
#61302=CARTESIAN_POINT ( 'NONE',  ( -111.4277742342994770, -292.2138600974926703, -251.6038216787700037 ) ) ;
#61303=CARTESIAN_POINT ( 'NONE',  ( -106.8196575601372160, -292.2811587237740127, -238.2018574513158455 ) ) ;
#61304=CARTESIAN_POINT ( 'NONE',  ( -42.39184327807954844, -294.9509342211956664, -343.1862239466129267 ) ) ;
#61305=CARTESIAN_POINT ( 'NONE',  ( 35.94504206854879413, -289.3476537100062274, -254.4220442554704960 ) ) ;
#61306=CARTESIAN_POINT ( 'NONE',  ( 21.06471466625051292, -281.0413661851348479, -220.1644744070667628 ) ) ;
#61307=CARTESIAN_POINT ( 'NONE',  ( -112.5131537814035596, -294.5344638699883717, -278.0140097385419153 ) ) ;
#61308=CARTESIAN_POINT ( 'NONE',  ( -4.165758162109444385, -282.4600952944311416, -339.8619859655595974 ) ) ;
#61309=CARTESIAN_POINT ( 'NONE',  ( 37.22871072067736264, -277.4760285213617976, -266.0187067795313851 ) ) ;
#61311=CARTESIAN_POINT ( 'NONE',  ( -25.97897899706188696, -275.0485102041932919, -345.2690217507361012 ) ) ;
#61313=CARTESIAN_POINT ( 'NONE',  ( -48.34413205242784528, -282.7036278771045090, -342.5894706792235525 ) ) ;
#61314=CARTESIAN_POINT ( 'NONE',  ( -82.01977402536080319, -280.6629638597428311, -208.1366980945376213 ) ) ;
#61315=CARTESIAN_POINT ( 'NONE',  ( 22.21498129637733854, -287.2629107389572596, -318.8154868346142621 ) ) ;
#61316=CARTESIAN_POINT ( 'NONE',  ( -19.85417759692977313, -294.0400414178182018, -198.3903920338735247 ) ) ;
#61317=CARTESIAN_POINT ( 'NONE',  ( 17.49953028613967021, -276.4195405220847874, -217.3809546641495558 ) ) ;
#61318=CARTESIAN_POINT ( 'NONE',  ( 38.64980932666259861, -276.9845087851921335, -279.6711557744969241 ) ) ;
#61319=CARTESIAN_POINT ( 'NONE',  ( -71.65606146089955075, -277.3521719186881569, -334.8075436313520186 ) ) ;
#61320=CARTESIAN_POINT ( 'NONE',  ( -78.54207375752608300, -299.4966662501169594, -207.8283818438405035 ) ) ;
#61321=CARTESIAN_POINT ( 'NONE',  ( -90.95908084453942877, -283.2891324060518627, -218.0832887304998735 ) ) ;
#61322=CARTESIAN_POINT ( 'NONE',  ( 38.83160638164084588, -293.0754463219067247, -258.8960487176551055 ) ) ;
#61323=CARTESIAN_POINT ( 'NONE',  ( -51.51630576280037843, -290.8306627055935678, -345.2311451536955360 ) ) ;
#61324=CARTESIAN_POINT ( 'NONE',  ( -30.76561074184070321, -291.0575578014143048, -197.3475499146429399 ) ) ;
#61326=CARTESIAN_POINT ( 'NONE',  ( 3.839378203651969024, -291.1692602114912916, -205.9343876785895020 ) ) ;
#61327=CARTESIAN_POINT ( 'NONE',  ( 12.92078424213064913, -292.4444249347257596, -217.3915970138668001 ) ) ;
#61329=CARTESIAN_POINT ( 'NONE',  ( -37.48714727442480665, -290.1335623523838763, -347.0648889991185229 ) ) ;
#61330=CARTESIAN_POINT ( 'NONE',  ( -110.4534051396120446, -279.2358177885050168, -267.9131134802931342 ) ) ;
#61332=CARTESIAN_POINT ( 'NONE',  ( -99.66230709163096435, -296.0671678049372986, -225.6662138221333294 ) ) ;
#61333=CARTESIAN_POINT ( 'NONE',  ( -43.66616751021834375, -286.6257701435818035, -193.6703801939447374 ) ) ;
#61334=CARTESIAN_POINT ( 'NONE',  ( -3.502480597322533917, -286.8199143526628063, -201.2043388997380191 ) ) ;
#61335=CARTESIAN_POINT ( 'NONE',  ( -90.75403265264685615, -284.1695977731365019, -320.1527861718582813 ) ) ;
#61336=CARTESIAN_POINT ( 'NONE',  ( 5.351633954136511662, -58.18680328362809462, -354.6685698517738956 ) ) ;
#61337=CARTESIAN_POINT ( 'NONE',  ( 178.3994555490664595, 253.9822658848526657, -165.8744343721958785 ) ) ;
#61338=CARTESIAN_POINT ( 'NONE',  ( -110.4036248592226883, -268.2063041062111779, -295.2719097700364159 ) ) ;
#61341=CARTESIAN_POINT ( 'NONE',  ( -64.40235718648879981, -276.6116120984796680, -338.3878774470868507 ) ) ;
#61342=CARTESIAN_POINT ( 'NONE',  ( -1.330328075974988478, -275.4832278153446623, -334.2731347728691844 ) ) ;
#61343=CARTESIAN_POINT ( 'NONE',  ( -51.78291062434480807, -297.3799286863383600, -194.7358077258001003 ) ) ;
#61344=CARTESIAN_POINT ( 'NONE',  ( -54.25878813547573287, -170.2527245721807674, -361.3251189563821981 ) ) ;
#61345=CARTESIAN_POINT ( 'NONE',  ( -92.98689987490215003, -276.5147790370451162, -322.9434431916723156 ) ) ;
#61346=CARTESIAN_POINT ( 'NONE',  ( -98.69559955160239895, -274.8808547389016326, -228.8731122167084493 ) ) ;
#61349=CARTESIAN_POINT ( 'NONE',  ( -110.1834597593814351, -290.9617243231936072, -276.6414324256516011 ) ) ;
#61350=CARTESIAN_POINT ( 'NONE',  ( -29.09146248775674692, -298.9558089973359074, -193.5215010717849964 ) ) ;
#61351=CARTESIAN_POINT ( 'NONE',  ( -112.5416896459395417, -297.2487730923247113, -254.0365000909214359 ) ) ;
#61352=CARTESIAN_POINT ( 'NONE',  ( -67.29326840376492669, -295.6228645130847781, -336.9473674665405838 ) ) ;
#61354=CARTESIAN_POINT ( 'NONE',  ( -109.2878775550504429, -280.1745326767582469, -293.6175345735392739 ) ) ;
#61355=CARTESIAN_POINT ( 'NONE',  ( -8.068112327127085592, -282.1866345898757231, -341.5694470780718461 ) ) ;
#61356=CARTESIAN_POINT ( 'NONE',  ( -41.85916117406565462, -278.0516909924560878, -343.4695893313004262 ) ) ;
#61357=CARTESIAN_POINT ( 'NONE',  ( 38.61161238814129604, -277.3580691624371752, -273.9731442986214347 ) ) ;
#61358=CARTESIAN_POINT ( 'NONE',  ( -111.0343129463638547, -271.0682070554903476, -267.5920783070110360 ) ) ;
#61360=CARTESIAN_POINT ( 'NONE',  ( -100.5817726090219963, -278.2176230215943065, -306.9275952081090395 ) ) ;
#61361=CARTESIAN_POINT ( 'NONE',  ( -13.12309273342502003, -275.1618187473196713, -197.4391194084294625 ) ) ;
#61362=CARTESIAN_POINT ( 'NONE',  ( 35.90836172644844737, -286.5164785535055785, -292.4911209200318467 ) ) ;
#61363=CARTESIAN_POINT ( 'NONE',  ( -73.01659179066888328, -275.5799314223348802, -204.3313919983325491 ) ) ;
#61364=CARTESIAN_POINT ( 'NONE',  ( 21.26691320780884453, -274.7917814940661287, -319.3880160849798813 ) ) ;
#61366=CARTESIAN_POINT ( 'NONE',  ( -90.71755185143608458, -289.0302182399763069, -320.4713006811011837 ) ) ;
#61367=CARTESIAN_POINT ( 'NONE',  ( -113.7174336871463396, -284.0127916790894460, -261.4134864651146017 ) ) ;
#61368=CARTESIAN_POINT ( 'NONE',  ( 3.937045986351015880, -280.7281057818884733, -331.8563086408301501 ) ) ;
#61369=CARTESIAN_POINT ( 'NONE',  ( 29.51554515754934727, -279.7139326480127579, -239.4902141343162612 ) ) ;
#61370=CARTESIAN_POINT ( 'NONE',  ( -111.7479600948059328, -282.6609840543524683, -268.1199859514173909 ) ) ;
#61371=CARTESIAN_POINT ( 'NONE',  ( 18.45970729333602023, -290.2506100977726078, -320.4919304166546112 ) ) ;
#61372=CARTESIAN_POINT ( 'NONE',  ( -101.1646098885806708, -280.2509444133464740, -234.1151982997666039 ) ) ;
#61374=CARTESIAN_POINT ( 'NONE',  ( 23.12505890027613731, -279.3267916984418662, -223.9694224978204602 ) ) ;
#61375=CARTESIAN_POINT ( 'NONE',  ( -19.87785883529945963, -294.2766665372810735, -197.3692922573578414 ) ) ;
#61376=CARTESIAN_POINT ( 'NONE',  ( -96.02041585157451209, -277.4494121126649588, -222.0627145472533073 ) ) ;
#61377=CARTESIAN_POINT ( 'NONE',  ( -45.91182601263462715, -277.8149640871089332, -343.0096489186244071 ) ) ;
#61378=CARTESIAN_POINT ( 'NONE',  ( -68.40499038298966639, -285.4594106739762083, -338.8229797264590388 ) ) ;
#61379=LINE ( 'NONE', #40940, #5056 ) ;
#61380=CARTESIAN_POINT ( 'NONE',  ( -68.73626708208199432, -291.3817169367707720, -339.1044142728047177 ) ) ;
#61381=CARTESIAN_POINT ( 'NONE',  ( 36.98561309977826994, -286.9937232199565642, -289.8446836032106262 ) ) ;
#61382=CARTESIAN_POINT ( 'NONE',  ( -94.04153049951951004, -289.6152080190131528, -223.1019042607424865 ) ) ;
#61384=CARTESIAN_POINT ( 'NONE',  ( 33.99185867087999213, -274.0051692665829819, -252.6759018827022771 ) ) ;
#61385=CARTESIAN_POINT ( 'NONE',  ( -7.513373677495008174, -292.7964785155708682, -338.3538637370785409 ) ) ;
#61388=CARTESIAN_POINT ( 'NONE',  ( 17.00948576330940298, -291.2891394793577433, -216.7268545940153217 ) ) ;
#61389=CARTESIAN_POINT ( 'NONE',  ( -84.17106336680740242, -286.9962781486806875, -213.2556727458677130 ) ) ;
#61390=CARTESIAN_POINT ( 'NONE',  ( 22.47570041525208140, -286.4269637230739818, -317.2419871467597545 ) ) ;
#61392=CARTESIAN_POINT ( 'NONE',  ( -40.01334061122588537, -287.4432019572795980, -196.8203996320497708 ) ) ;
#61393=CARTESIAN_POINT ( 'NONE',  ( 115.2448031289451222, -299.5541904835127980, -198.8526868767648352 ) ) ;
#61394=CARTESIAN_POINT ( 'NONE',  ( 33.54247527635438075, -288.1158489833282488, -252.1988328905676724 ) ) ;
#61395=CARTESIAN_POINT ( 'NONE',  ( 37.60405666649064216, -295.6384516039051960, -278.6875295515017115 ) ) ;
#61396=CARTESIAN_POINT ( 'NONE',  ( -95.06524177541561471, -275.9624327789842368, -319.1387311271998328 ) ) ;
#61397=CARTESIAN_POINT ( 'NONE',  ( -87.07829578468785314, -278.0559330804764500, -329.1847129839409263 ) ) ;
#61398=CARTESIAN_POINT ( 'NONE',  ( -50.29499807841217773, -289.9678772898131456, -195.9196895457591268 ) ) ;
#61399=CARTESIAN_POINT ( 'NONE',  ( -64.74232811921139330, -279.7041910848450357, -198.3451387244329283 ) ) ;
#61400=CARTESIAN_POINT ( 'NONE',  ( -35.79761705321728726, -300.0514629402524065, -195.7157852367089390 ) ) ;
#61402=CARTESIAN_POINT ( 'NONE',  ( -111.8629285205952897, -282.4375830952704405, -279.2713490570718591 ) ) ;
#61404=CARTESIAN_POINT ( 'NONE',  ( -108.8009961343364012, -276.9536952206743763, -250.2035018576559935 ) ) ;
#61405=CARTESIAN_POINT ( 'NONE',  ( 18.28262132308068288, -280.2540963088529224, -320.7454723108579628 ) ) ;
#61406=CARTESIAN_POINT ( 'NONE',  ( -75.01093283198058259, -276.0244077164914529, -336.7217739507690339 ) ) ;
#61408=CARTESIAN_POINT ( 'NONE',  ( -73.62709049711578757, -297.0632615374768193, -334.5021984130257238 ) ) ;
#61409=CARTESIAN_POINT ( 'NONE',  ( -67.77139653902742111, -282.3625946972241536, -340.7566156138795463 ) ) ;
#61410=CARTESIAN_POINT ( 'NONE',  ( -98.65109707473668266, -298.0478409866923357, -230.2122883406818232 ) ) ;
#61411=CARTESIAN_POINT ( 'NONE',  ( -77.95495267552034591, -298.8336284172539195, -205.5239219474385663 ) ) ;
#61412=CARTESIAN_POINT ( 'NONE',  ( 20.70092020750152884, -274.5957205646369061, -226.0331798433515758 ) ) ;
#61413=CARTESIAN_POINT ( 'NONE',  ( 5.629242589961247489, -294.6339370983061485, -208.8279753140617743 ) ) ;
#61414=CARTESIAN_POINT ( 'NONE',  ( 38.10871369454270052, -287.9110536380823646, -285.7310580775337030 ) ) ;
#61415=CARTESIAN_POINT ( 'NONE',  ( 2.826228734243690255, -274.6592971622505388, -334.6633726329814067 ) ) ;
#61416=CARTESIAN_POINT ( 'NONE',  ( -74.42918108061037685, -289.3646693668756598, -337.8559372751926730 ) ) ;
#61418=CARTESIAN_POINT ( 'NONE',  ( 25.15774563281336995, -286.0866525304282959, -232.1874657156944295 ) ) ;
#61419=CARTESIAN_POINT ( 'NONE',  ( -109.3057593288156113, -288.8240063711422749, -249.2382670070191466 ) ) ;
#61421=CARTESIAN_POINT ( 'NONE',  ( 88.37812178648184158, 82.46720509654242903, -304.8213980281626618 ) ) ;
#61422=CARTESIAN_POINT ( 'NONE',  ( -73.58093152415898430, -289.0546347464799624, -333.8161171322937548 ) ) ;
#61424=CARTESIAN_POINT ( 'NONE',  ( -85.94411423481727752, -284.6481988035160384, -329.7801852529115081 ) ) ;
#61425=CARTESIAN_POINT ( 'NONE',  ( 29.27740950945138110, -292.1138533835527937, -232.2203990129869737 ) ) ;
#61426=CARTESIAN_POINT ( 'NONE',  ( 37.46538932571372982, -282.9689897271921950, -255.8580222907608288 ) ) ;
#61427=CARTESIAN_POINT ( 'NONE',  ( -19.88512593388098892, -281.5870419396055695, -195.8180022544659096 ) ) ;
#61428=CARTESIAN_POINT ( 'NONE',  ( -61.53672519101359484, -283.2085972770206013, -339.2881580002921851 ) ) ;
#61429=CARTESIAN_POINT ( 'NONE',  ( 24.11904343356764713, -278.1367644770287484, -313.4337773170307742 ) ) ;
#61430=CARTESIAN_POINT ( 'NONE',  ( -107.7730309721822124, -296.9506773564249897, -239.1097205282081291 ) ) ;
#61431=CARTESIAN_POINT ( 'NONE',  ( -51.67391808818965870, -275.1802827099421052, -198.2268631980161047 ) ) ;
#61432=CARTESIAN_POINT ( 'NONE',  ( -6.569656479832156393, -290.4783527478678593, -202.3542937983152683 ) ) ;
#61433=CARTESIAN_POINT ( 'NONE',  ( -99.60927132711695720, -271.8805023964864631, -231.5039425651470424 ) ) ;
#61434=ORIENTED_EDGE ( 'NONE', *, *, #44228, .T. ) ;
#61436=CARTESIAN_POINT ( 'NONE',  ( -102.2588566181382106, -286.9623344743721987, -233.8263512287691697 ) ) ;
#61437=CARTESIAN_POINT ( 'NONE',  ( 6.448821540586438417, -295.5524777293240959, -333.3852067386901581 ) ) ;
#61438=CARTESIAN_POINT ( 'NONE',  ( -74.77942668136779503, -286.1908312449459686, -207.5733062774455107 ) ) ;
#61440=CARTESIAN_POINT ( 'NONE',  ( -22.99466727141519229, -275.9318096968128202, -345.8272230398811189 ) ) ;
#61441=CARTESIAN_POINT ( 'NONE',  ( -13.90542449179094930, -292.9997356293948769, -197.0655184142523240 ) ) ;
#61442=CARTESIAN_POINT ( 'NONE',  ( 37.08138574416904731, -285.5113130251838811, -256.1657042154923829 ) ) ;
#61443=CARTESIAN_POINT ( 'NONE',  ( -25.02900512212269746, -292.5383591334406219, -194.3733437478906012 ) ) ;
#61444=CARTESIAN_POINT ( 'NONE',  ( -72.36527503667066696, -289.8625635077495417, -334.4347996891973480 ) ) ;
#61446=CARTESIAN_POINT ( 'NONE',  ( -82.33893616535382876, -218.9925579527750301, -348.9763288427828343 ) ) ;
#61447=CARTESIAN_POINT ( 'NONE',  ( -68.23793463958713801, -287.1738228914134652, -200.5748802341978489 ) ) ;
#61448=CARTESIAN_POINT ( 'NONE',  ( -99.86837403722181250, -276.6952119285918457, -220.4570493818173702 ) ) ;
#61450=CARTESIAN_POINT ( 'NONE',  ( 22.37323797389218072, -279.8809646230564567, -227.8363929208654781 ) ) ;
#61451=CARTESIAN_POINT ( 'NONE',  ( -112.0643677754729595, -278.4509914101101913, -251.8065837479296363 ) ) ;
#61452=CARTESIAN_POINT ( 'NONE',  ( -75.46107267245471917, -281.5430959746002486, -205.9047935234524971 ) ) ;
#61453=CARTESIAN_POINT ( 'NONE',  ( -104.7603843068534104, -262.4557100720102767, -316.6309476432972474 ) ) ;
#61454=CARTESIAN_POINT ( 'NONE',  ( 24.61877116015681466, -280.7246355570950413, -315.0991609931664925 ) ) ;
#61455=CARTESIAN_POINT ( 'NONE',  ( -24.84211793245598443, -284.2323434094514596, -196.7178524456427908 ) ) ;
#61456=CARTESIAN_POINT ( 'NONE',  ( -23.61084004444499485, -299.9819473029384085, -194.3703956122839998 ) ) ;
#61457=CARTESIAN_POINT ( 'NONE',  ( -55.81281796273394491, -295.7886654723936317, -341.1016354192264544 ) ) ;
#61459=CARTESIAN_POINT ( 'NONE',  ( -5.814994546087259408, -291.1603951620834323, -203.9596646753071809 ) ) ;
#61460=CARTESIAN_POINT ( 'NONE',  ( 37.14208259394408174, -276.4431242236773301, -289.4786203918422984 ) ) ;
#61461=CARTESIAN_POINT ( 'NONE',  ( 30.17481857447199545, -275.1785295998173524, -242.4701479630790857 ) ) ;
#61462=CARTESIAN_POINT ( 'NONE',  ( 19.81472236261294739, -273.7755261625891308, -219.1495490646263988 ) ) ;
#61464=CARTESIAN_POINT ( 'NONE',  ( -58.11829912362318140, -271.7836733630734329, -198.2428810843090048 ) ) ;
#61466=CARTESIAN_POINT ( 'NONE',  ( -44.72051730037452444, -296.5689367847056701, -346.4677762402475878 ) ) ;
#61469=CARTESIAN_POINT ( 'NONE',  ( -96.16157294211976136, -285.0206594225489880, -314.1155307486350807 ) ) ;
#61470=CARTESIAN_POINT ( 'NONE',  ( 38.51907482650000958, -283.3782910712143348, -275.5688201612044281 ) ) ;
#61471=CARTESIAN_POINT ( 'NONE',  ( -105.6572487490586241, -284.2476244511596519, -244.3442295329869012 ) ) ;
#61472=CARTESIAN_POINT ( 'NONE',  ( -81.31217839892325117, -276.0612432209869098, -329.6319999886777623 ) ) ;
#61473=CARTESIAN_POINT ( 'NONE',  ( -23.81761041706950266, -284.7379508881656420, -343.3540250022544456 ) ) ;
#61474=CARTESIAN_POINT ( 'NONE',  ( -96.66252507877891276, -276.4247662693406937, -314.1058112127864774 ) ) ;
#61475=CARTESIAN_POINT ( 'NONE',  ( 21.72210377702268858, -276.0259536602487742, -226.9365495615540169 ) ) ;
#61476=CARTESIAN_POINT ( 'NONE',  ( -113.5582899549025058, -279.4823359841267916, -260.1993774051363175 ) ) ;
#61479=CARTESIAN_POINT ( 'NONE',  ( -96.62889079012583693, -287.0543867561888760, -223.1876666720501987 ) ) ;
#61480=CARTESIAN_POINT ( 'NONE',  ( -50.51028373539165273, -294.4218007088908280, -342.3277083718405152 ) ) ;
#61481=CARTESIAN_POINT ( 'NONE',  ( -95.38681836540783365, -289.2180863572851308, -320.7999624938732381 ) ) ;
#61482=CARTESIAN_POINT ( 'NONE',  ( 18.23300165627940217, -285.4447545129391983, -222.1239182315387382 ) ) ;
#61483=CARTESIAN_POINT ( 'NONE',  ( -97.57312137477052261, -289.3857976213455458, -227.2610938846886199 ) ) ;
#61484=CARTESIAN_POINT ( 'NONE',  ( -67.93596766645501361, -284.6680758788762660, -337.0778422711407529 ) ) ;
#61485=CARTESIAN_POINT ( 'NONE',  ( 20.17989833638084107, -274.2169863135529795, -318.4887229749992912 ) ) ;
#61486=CARTESIAN_POINT ( 'NONE',  ( -62.91358121270257442, -284.1245327268627534, -198.5800667750541209 ) ) ;
#61487=CARTESIAN_POINT ( 'NONE',  ( 36.32092951419483029, -289.3712653618989634, -256.2608468642360435 ) ) ;
#61488=CARTESIAN_POINT ( 'NONE',  ( 18.93158292204115156, -284.8598328238511499, -220.4510693306722828 ) ) ;
#61489=CARTESIAN_POINT ( 'NONE',  ( 24.33505303338034764, -283.0390337919583885, -309.9434359571995969 ) ) ;
#61490=CARTESIAN_POINT ( 'NONE',  ( -73.52197408791941768, -291.5311599035569543, -336.2621993457808571 ) ) ;
#61493=CARTESIAN_POINT ( 'NONE',  ( -94.47631268537686822, -297.7915505840637138, -319.8075561569701222 ) ) ;
#61494=CARTESIAN_POINT ( 'NONE',  ( 1.455780395478187828, -278.5700010461696934, -206.1156628961948059 ) ) ;
#61495=CARTESIAN_POINT ( 'NONE',  ( 36.55169625369870801, -292.4841139265116681, -249.2436295050563331 ) ) ;
#61496=CARTESIAN_POINT ( 'NONE',  ( -97.52343850647956458, -295.5420461995283858, -227.6457954173676512 ) ) ;
#61497=CARTESIAN_POINT ( 'NONE',  ( 31.53832800146757265, -279.8957251927471361, -244.5872050574532466 ) ) ;
#61498=CARTESIAN_POINT ( 'NONE',  ( 26.52360592865664657, -273.1149907170185429, -232.0180952566425390 ) ) ;
#61499=CARTESIAN_POINT ( 'NONE',  ( 36.20156353142176897, -294.8723754790291878, -270.7459023020772975 ) ) ;
#61501=CARTESIAN_POINT ( 'NONE',  ( -110.4678789762892990, -271.4092890200255965, -248.0180792343690541 ) ) ;
#61502=CARTESIAN_POINT ( 'NONE',  ( -32.10501939145949279, -293.2268402529552986, -346.1802083345339724 ) ) ;
#61503=CARTESIAN_POINT ( 'NONE',  ( 29.26417206702861407, -294.5567129385108842, -238.9514180124777170 ) ) ;
#61504=DIRECTION ( 'NONE',  ( -1.000000000000000000, -0.000000000000000000, -0.000000000000000000 ) ) ;
#61505=CARTESIAN_POINT ( 'NONE',  ( 33.93505744973376892, -294.5728157658050463, -286.9156028189549943 ) ) ;
#61507=CARTESIAN_POINT ( 'NONE',  ( -8.688179225933367889, -280.6993297854849629, -340.1113648317503362 ) ) ;
#61508=CARTESIAN_POINT ( 'NONE',  ( -3.143756393969438179, -294.5870452864601248, -334.8553087624939053 ) ) ;
#61509=CARTESIAN_POINT ( 'NONE',  ( 28.30500385160923926, -282.0790964816146698, -310.7053016491167909 ) ) ;
#61510=CARTESIAN_POINT ( 'NONE',  ( -76.75071982764404765, -283.2309225159081052, -336.5491155393883105 ) ) ;
#61511=CARTESIAN_POINT ( 'NONE',  ( -112.2011284414167989, -288.5773692399648667, -268.3886428612408395 ) ) ;
#61513=CARTESIAN_POINT ( 'NONE',  ( 37.00639391132412470, -279.8146009653883652, -253.1260813463499630 ) ) ;
#61514=CARTESIAN_POINT ( 'NONE',  ( 14.38503507160792161, -287.2656527834864733, -327.0531835923711697 ) ) ;
#61516=CARTESIAN_POINT ( 'NONE',  ( -10.17677864706474722, -296.2916617261439001, -338.9796829379534415 ) ) ;
#61517=CARTESIAN_POINT ( 'NONE',  ( -70.03232798151306326, -278.8995801838204898, -339.4401173282693094 ) ) ;
#61518=CARTESIAN_POINT ( 'NONE',  ( -57.11486062434031652, -279.4566356340969833, -200.0680912254142925 ) ) ;
#61519=CARTESIAN_POINT ( 'NONE',  ( 11.11714006095851204, -292.8683760509114791, -210.4532291340083532 ) ) ;
#61520=CARTESIAN_POINT ( 'NONE',  ( -104.5153971260959480, -282.1762925267153150, -305.0731624576172862 ) ) ;
#61521=CARTESIAN_POINT ( 'NONE',  ( -69.42180986089981332, -279.4743752147767282, -338.1680043409789391 ) ) ;
#61522=CARTESIAN_POINT ( 'NONE',  ( 24.61995384112986684, -293.1496043309717265, -309.4968696820446894 ) ) ;
#61523=CARTESIAN_POINT ( 'NONE',  ( -83.95301859143829404, -295.4115979741238220, -211.6041129812376482 ) ) ;
#61526=CARTESIAN_POINT ( 'NONE',  ( -9.212978297705529229, -294.1818684772928236, -337.8044273669349309 ) ) ;
#61528=CARTESIAN_POINT ( 'NONE',  ( 27.33386217378598815, -291.4809262143062369, -301.5434626090942629 ) ) ;
#61529=CARTESIAN_POINT ( 'NONE',  ( -114.1802237732302387, -271.7494487974028061, -270.3509185704776883 ) ) ;
#61530=CARTESIAN_POINT ( 'NONE',  ( 23.61233811165435270, -279.0840084129175693, -225.3621101606552770 ) ) ;
#61531=CARTESIAN_POINT ( 'NONE',  ( -78.27285679202557844, -286.8289287694049108, -205.7241418291234538 ) ) ;
#61532=CARTESIAN_POINT ( 'NONE',  ( -42.66603306456350708, -288.9543693118744159, -343.2172950924804695 ) ) ;
#61533=CARTESIAN_POINT ( 'NONE',  ( -89.56361126698323005, -279.3244425694189772, -322.4295198765239547 ) ) ;
#61534=CARTESIAN_POINT ( 'NONE',  ( -110.6830428665489450, -274.2594826906876619, -262.1460184820764425 ) ) ;
#61535=CARTESIAN_POINT ( 'NONE',  ( -48.68426251022908957, -275.9945798105036374, -342.9281435129106512 ) ) ;
#61537=CARTESIAN_POINT ( 'NONE',  ( -37.60332984904555076, -297.7156808445990919, -193.3827064533411146 ) ) ;
#61538=CARTESIAN_POINT ( 'NONE',  ( -109.8353161666531292, -292.6917963651112018, -253.3942188511090876 ) ) ;
#61539=CARTESIAN_POINT ( 'NONE',  ( 6.174032552145646946, -296.0728509225353378, -332.9779720756002916 ) ) ;
#61541=CARTESIAN_POINT ( 'NONE',  ( -109.8896582381250937, -291.0852390379755548, -279.3436812136667982 ) ) ;
#61543=CARTESIAN_POINT ( 'NONE',  ( 38.21112658040112109, -291.6197507629605639, -264.6975630184206238 ) ) ;
#61544=CARTESIAN_POINT ( 'NONE',  ( -43.29235780551449864, -298.3123637854193362, -193.5594111415594227 ) ) ;
#61545=CARTESIAN_POINT ( 'NONE',  ( -105.8241808029595745, -296.5584312415042518, -244.8728916037269698 ) ) ;
#61548=CARTESIAN_POINT ( 'NONE',  ( -112.9815466882613606, -292.2041933408694376, -259.9077001395103821 ) ) ;
#61549=CARTESIAN_POINT ( 'NONE',  ( -86.96033596737727578, -287.3602571626767030, -214.2738096480571528 ) ) ;
#61550=CARTESIAN_POINT ( 'NONE',  ( -51.89363856869665170, -271.8654817022522252, -196.9031983860462844 ) ) ;
#61551=CARTESIAN_POINT ( 'NONE',  ( -13.62944216140255982, -276.2825356963100489, -199.7987837056423643 ) ) ;
#61552=CARTESIAN_POINT ( 'NONE',  ( 26.08744408407482496, -291.1041843294155456, -231.3009497301416388 ) ) ;
#61553=CARTESIAN_POINT ( 'NONE',  ( -98.63629697510526739, -279.8117827392970298, -314.9171776963686966 ) ) ;
#61555=CARTESIAN_POINT ( 'NONE',  ( 24.21179613797572827, -281.4466253359879602, -309.8884051730248643 ) ) ;
#61556=CARTESIAN_POINT ( 'NONE',  ( -88.99374129097709840, -278.8379479188694177, -327.0493809011744588 ) ) ;
#61557=CARTESIAN_POINT ( 'NONE',  ( -28.25678522229615908, -278.9597868732846564, -194.2454716615108907 ) ) ;
#61558=CARTESIAN_POINT ( 'NONE',  ( -84.40583500399526429, -218.0948329967893642, -349.5577229382324163 ) ) ;
#61559=CARTESIAN_POINT ( 'NONE',  ( 9.357681950251764746, -275.6177469845693508, -209.4350322245835514 ) ) ;
#61561=CARTESIAN_POINT ( 'NONE',  ( 6.817839845103098817, -276.1606719208120353, -208.0657226290591950 ) ) ;
#61562=CARTESIAN_POINT ( 'NONE',  ( -95.95921662488163406, -298.4090924074130271, -317.1477375740089997 ) ) ;
#61565=CARTESIAN_POINT ( 'NONE',  ( -95.18601776173989037, -290.9997319683336627, -315.4176125127284536 ) ) ;
#61566=CARTESIAN_POINT ( 'NONE',  ( 13.55133964658240053, -288.5130015190085260, -213.8647306276573374 ) ) ;
#61567=CARTESIAN_POINT ( 'NONE',  ( -68.80936241708438672, -288.8257457813284645, -336.3435315383437114 ) ) ;
#61568=CARTESIAN_POINT ( 'NONE',  ( -29.46300093431857903, -285.6570733878498345, -193.8271189874319020 ) ) ;
#61570=CARTESIAN_POINT ( 'NONE',  ( 34.85200946160615132, -279.7514410338675930, -254.9871473504247774 ) ) ;
#61571=CARTESIAN_POINT ( 'NONE',  ( 28.74718094033504556, -288.9594990387930693, -236.4377144467182177 ) ) ;
#61572=CARTESIAN_POINT ( 'NONE',  ( 1.449971091069490958, -281.0038303665621697, -333.0778106514468959 ) ) ;
#61573=CARTESIAN_POINT ( 'NONE',  ( -109.5244966888453888, -279.6854236707175687, -284.2437333962120078 ) ) ;
#61574=CARTESIAN_POINT ( 'NONE',  ( 0.6134218090894920650, -289.5006452849897300, -337.1462158489534318 ) ) ;
#61575=CARTESIAN_POINT ( 'NONE',  ( -95.31802922739805695, -278.4195060548344713, -314.8215915070111350 ) ) ;
#61576=CARTESIAN_POINT ( 'NONE',  ( -111.5412756187544261, -289.1070073158556397, -289.4512742759040975 ) ) ;
#61577=CARTESIAN_POINT ( 'NONE',  ( -105.2940793232880026, -285.8203593148964501, -234.3774983283701090 ) ) ;
#61578=CARTESIAN_POINT ( 'NONE',  ( -32.31670539856073532, -286.6062361674736962, -193.5737716788744081 ) ) ;
#61579=CARTESIAN_POINT ( 'NONE',  ( -109.4214679451498853, -284.8723010540758196, -258.7273982196827546 ) ) ;
#61582=CARTESIAN_POINT ( 'NONE',  ( -112.8789282410077561, -292.3298204791718717, -276.8714205272397635 ) ) ;
#61583=CARTESIAN_POINT ( 'NONE',  ( 35.89271610987277228, -292.5186696272881477, -292.6768108312361392 ) ) ;
#61584=CARTESIAN_POINT ( 'NONE',  ( 34.93740733541853416, -274.7700269064890790, -282.4629565876073229 ) ) ;
#61585=CARTESIAN_POINT ( 'NONE',  ( -114.2074343173303248, -295.9461899181725926, -266.7318064453463649 ) ) ;
#61586=CARTESIAN_POINT ( 'NONE',  ( -88.39711606821805390, -289.8010988518086037, -217.1488024720823375 ) ) ;
#61587=CARTESIAN_POINT ( 'NONE',  ( -7.601414920228121375, -292.8967370202886400, -338.1501680024688312 ) ) ;
#61588=CARTESIAN_POINT ( 'NONE',  ( -110.5172093716584953, -291.6743380765848315, -276.6792795940152132 ) ) ;
#61590=CARTESIAN_POINT ( 'NONE',  ( 35.31713995567030651, -291.3044901842745276, -251.0572673468768983 ) ) ;
#61591=CARTESIAN_POINT ( 'NONE',  ( -91.39072905797685564, -297.8208941614880700, -322.4320005777087772 ) ) ;
#61592=CARTESIAN_POINT ( 'NONE',  ( 35.78681571125072480, -288.4302701689059063, -265.5593704035121050 ) ) ;
#61593=CARTESIAN_POINT ( 'NONE',  ( 29.10488408497458579, -278.0026853319333782, -306.0137065524402260 ) ) ;
#61594=CARTESIAN_POINT ( 'NONE',  ( -110.2932645535070151, -277.0498069350354058, -293.9003250733066466 ) ) ;
#61595=CARTESIAN_POINT ( 'NONE',  ( -95.44227462878096446, -296.4307105408476559, -219.9977073298028927 ) ) ;
#61596=CARTESIAN_POINT ( 'NONE',  ( 21.63093920567703776, -274.4119381339535835, -315.0847339572242731 ) ) ;
#61597=CARTESIAN_POINT ( 'NONE',  ( -32.85220798371379658, -278.1890079382548606, -196.0566183925323855 ) ) ;
#61598=CARTESIAN_POINT ( 'NONE',  ( 19.29552080841105166, -276.0991754117393384, -223.6775479536968874 ) ) ;
#61599=CARTESIAN_POINT ( 'NONE',  ( -17.58515827736567516, -275.2012800044492451, -343.9554076225475114 ) ) ;
#61600=DIRECTION ( 'NONE',  ( 1.000000000000000000, 0.000000000000000000, 0.000000000000000000 ) ) ;
#61601=CARTESIAN_POINT ( 'NONE',  ( -36.49128131194280655, -298.8659001945193836, -197.1995205611631263 ) ) ;
#61603=CARTESIAN_POINT ( 'NONE',  ( 17.43157566775478173, -286.2944982594826229, -322.1133649038514477 ) ) ;
#61604=CARTESIAN_POINT ( 'NONE',  ( -34.03855549380171652, -273.9281724191407648, -197.4358875060958667 ) ) ;
#61605=CARTESIAN_POINT ( 'NONE',  ( -34.66682091908305097, -289.0194085136268427, -347.3146430559266946 ) ) ;
#61606=CARTESIAN_POINT ( 'NONE',  ( 95.53882501024096996, -301.6877222252096544, -194.9613191052525565 ) ) ;
#61607=CARTESIAN_POINT ( 'NONE',  ( -109.9476671421566323, -294.7858889351487619, -252.1868659936057497 ) ) ;
#61609=CARTESIAN_POINT ( 'NONE',  ( 1.301628852008377857, -279.7513899201317713, -203.8862910276628782 ) ) ;
#61610=EDGE_CURVE ( 'NONE', #9799, #78639, #1880, .T. ) ;
#61612=CARTESIAN_POINT ( 'NONE',  ( -79.18647895631424660, -277.4878362949309007, -208.0580722848341964 ) ) ;
#61614=CARTESIAN_POINT ( 'NONE',  ( -106.9429893934029110, -289.6548281415971360, -247.0632417422967819 ) ) ;
#61617=CARTESIAN_POINT ( 'NONE',  ( -112.3678546950538362, -288.5773692419674035, -268.3843062701905069 ) ) ;
#61618=CARTESIAN_POINT ( 'NONE',  ( -62.28238122372991370, -275.2418924425022055, -201.0165422859898854 ) ) ;
#61619=CARTESIAN_POINT ( 'NONE',  ( -21.82775345596143168, -284.2823426414564096, -345.1803919028450878 ) ) ;
#61620=CARTESIAN_POINT ( 'NONE',  ( 6.811864119086142644, -296.6223629286291157, -195.0207196009186532 ) ) ;
#61621=CARTESIAN_POINT ( 'NONE',  ( -110.3093251802722961, -284.5808290741047131, -268.1872517854639568 ) ) ;
#61622=CARTESIAN_POINT ( 'NONE',  ( -81.43848552385682638, -274.8646183644429470, -211.3832579355976691 ) ) ;
#61623=CARTESIAN_POINT ( 'NONE',  ( -38.09425688055099357, -274.8453181833588133, -197.2035115027000529 ) ) ;
#61624=CARTESIAN_POINT ( 'NONE',  ( -63.19798050311779747, -285.3891191477447933, -340.7632018540765557 ) ) ;
#61625=CARTESIAN_POINT ( 'NONE',  ( -47.29289401283886463, -296.9814875110316166, -197.7536808889494182 ) ) ;
#61627=CARTESIAN_POINT ( 'NONE',  ( 203.4918146885830481, 295.8998777880566422, -54.00000000006195933 ) ) ;
#61628=CARTESIAN_POINT ( 'NONE',  ( 37.76177754168008960, -293.1723935388689029, -253.3176585523507356 ) ) ;
#61629=CARTESIAN_POINT ( 'NONE',  ( -88.84725495041318766, -287.3042677641889213, -216.3331194698016589 ) ) ;
#61631=CARTESIAN_POINT ( 'NONE',  ( -37.30987171927208834, -271.5523547857346784, -190.3611179825600175 ) ) ;
#61632=CARTESIAN_POINT ( 'NONE',  ( -98.68070804685318365, -277.1314987317454097, -316.6610580569629292 ) ) ;
#61633=CARTESIAN_POINT ( 'NONE',  ( -110.4587335633697620, -289.2239738649168430, -248.9055863497066525 ) ) ;
#61634=CARTESIAN_POINT ( 'NONE',  ( 8.237837126473619875, -283.9360829183072497, -328.3332409107633225 ) ) ;
#61635=CARTESIAN_POINT ( 'NONE',  ( -101.4494962044501705, -279.8108276321997892, -307.4527048382374232 ) ) ;
#61636=CARTESIAN_POINT ( 'NONE',  ( 1.208609612536031275, -287.9816049563006572, -204.3725716139126973 ) ) ;
#61637=CARTESIAN_POINT ( 'NONE',  ( 32.93568061977403971, -283.2105256904349062, -244.0189320777680564 ) ) ;
#61638=CARTESIAN_POINT ( 'NONE',  ( 11.78406013720823964, -274.8791515353786963, -210.9988357890421753 ) ) ;
#61639=CARTESIAN_POINT ( 'NONE',  ( -93.33545199929558578, -277.6630877529099166, -323.2930920257721823 ) ) ;
#61640=CARTESIAN_POINT ( 'NONE',  ( -64.06351671530785552, -297.3234540689977621, -339.8942007019927587 ) ) ;
#61643=CARTESIAN_POINT ( 'NONE',  ( -4.062703894991550158, -296.6041284862747602, -194.6067220786430880 ) ) ;
#61644=CARTESIAN_POINT ( 'NONE',  ( -74.04961317085174244, -277.0618020572221667, -333.5316614481918123 ) ) ;
#61645=CARTESIAN_POINT ( 'NONE',  ( -38.36756563531905329, -275.2446298607903259, -193.7650585525773010 ) ) ;
#61646=CARTESIAN_POINT ( 'NONE',  ( 0.6701143928098732827, -288.3261633126162451, -206.7948747367249496 ) ) ;
#61647=CARTESIAN_POINT ( 'NONE',  ( -110.9183084765487735, -297.8165728502071374, -290.5895746169477434 ) ) ;
#61648=CARTESIAN_POINT ( 'NONE',  ( -96.19644211928942923, -297.0940644155557493, -319.4134174006304647 ) ) ;
#61649=CARTESIAN_POINT ( 'NONE',  ( -98.26847706228650736, -293.1454919964240275, -226.8228107717127955 ) ) ;
#61650=CARTESIAN_POINT ( 'NONE',  ( -90.76498441072926937, -277.2926712025489451, -217.8855981709258174 ) ) ;
#61651=CARTESIAN_POINT ( 'NONE',  ( 36.45713297567899502, -283.3412445047342771, -260.2296440644144013 ) ) ;
#61652=CARTESIAN_POINT ( 'NONE',  ( -111.5174836037884774, -270.6800391692093513, -262.0064817008655496 ) ) ;
#61653=CARTESIAN_POINT ( 'NONE',  ( -33.10376765255829667, -284.8597511755815503, -346.0202278069147042 ) ) ;
#61654=CARTESIAN_POINT ( 'NONE',  ( 35.42940636871686166, -286.5889295323000852, -279.2263383793293201 ) ) ;
#61655=CARTESIAN_POINT ( 'NONE',  ( -20.56528858298729290, -109.1840546197655470, -362.3597369185399657 ) ) ;
#61657=CARTESIAN_POINT ( 'NONE',  ( -25.13410883894809444, -285.8786893664658351, -198.3163175086395995 ) ) ;
#61659=CARTESIAN_POINT ( 'NONE',  ( -112.2202933879071054, -285.4237050203911394, -286.9348557239857769 ) ) ;
#61660=CARTESIAN_POINT ( 'NONE',  ( 8.971375338740864791, -299.1396686334033461, -197.2955806747803535 ) ) ;
#61661=CARTESIAN_POINT ( 'NONE',  ( 11.83448627258825425, -285.5123635919666185, -211.5576456572826771 ) ) ;
#61662=CARTESIAN_POINT ( 'NONE',  ( -8.959283811377348528, -281.3557079400586076, -199.0360967272378048 ) ) ;
#61664=CARTESIAN_POINT ( 'NONE',  ( -28.32630538649357277, -281.6845454442236587, -194.5357499768319940 ) ) ;
#61665=CARTESIAN_POINT ( 'NONE',  ( 15.14381404256942787, -281.1018422207299636, -213.9764870977493558 ) ) ;
#61666=CARTESIAN_POINT ( 'NONE',  ( -67.68488546085839630, -283.1237833571631768, -207.2794874003663779 ) ) ;
#61667=CARTESIAN_POINT ( 'NONE',  ( 45.84035832368225272, 12.14739099000767730, -332.1170644278120676 ) ) ;
#61669=CARTESIAN_POINT ( 'NONE',  ( 18.82777259319304264, -278.2412231372006772, -319.8275887456744613 ) ) ;
#61670=CARTESIAN_POINT ( 'NONE',  ( 153.2297941377568407, 207.2841453618251819, -217.1594761235724320 ) ) ;
#61671=CARTESIAN_POINT ( 'NONE',  ( 37.34829943842961342, -279.5851454590617209, -271.3603852724700687 ) ) ;
#61672=CARTESIAN_POINT ( 'NONE',  ( -7.607660556225663839, -294.1967127028186724, -200.4194464810985323 ) ) ;
#61673=CARTESIAN_POINT ( 'NONE',  ( -38.35201194435276051, -294.4137330658026599, -343.4560695084881559 ) ) ;
#61674=CARTESIAN_POINT ( 'NONE',  ( -112.2559168738368669, -290.2792572273092446, -252.8286614250167474 ) ) ;
#61675=PLANE ( 'NONE',  #76248 ) ;
#61676=CARTESIAN_POINT ( 'NONE',  ( -94.22516100884091372, -294.4291879782468868, -321.3990278339487077 ) ) ;
#61677=CARTESIAN_POINT ( 'NONE',  ( 34.49367532732674135, -285.7305907533730078, -253.3913801277508071 ) ) ;
#61678=CARTESIAN_POINT ( 'NONE',  ( 23.58843184267866633, -294.8310414569473323, -227.9313664620355837 ) ) ;
#61679=CARTESIAN_POINT ( 'NONE',  ( -108.5103788932554636, -286.1077729990337843, -252.0236524524885340 ) ) ;
#61681=CARTESIAN_POINT ( 'NONE',  ( 37.84257486308012375, -294.6878001315683377, -285.8577307696962748 ) ) ;
#61682=CARTESIAN_POINT ( 'NONE',  ( -84.89709012618668282, -284.2216005811472428, -325.8270834352526890 ) ) ;
#61683=CARTESIAN_POINT ( 'NONE',  ( -65.47204102606404774, -294.2067780506824874, -341.6261811681040399 ) ) ;
#61684=CARTESIAN_POINT ( 'NONE',  ( -112.1623766457083349, -291.5742273284855060, -252.8675423958449642 ) ) ;
#61685=CARTESIAN_POINT ( 'NONE',  ( -95.61841011882198416, -291.7235285240469125, -220.1080016883039150 ) ) ;
#61686=CARTESIAN_POINT ( 'NONE',  ( -23.78309366172603490, -289.0408803685299972, -342.1426170189960771 ) ) ;
#61689=CARTESIAN_POINT ( 'NONE',  ( -37.27878502387808624, -299.9133432668988348, -194.5955393664444841 ) ) ;
#61690=CARTESIAN_POINT ( 'NONE',  ( -107.7066562029457089, -271.7363077118395154, -239.9486306444150898 ) ) ;
#61691=CARTESIAN_POINT ( 'NONE',  ( 19.02485570723045427, -279.9497379580461711, -223.5846208274220146 ) ) ;
#61693=CARTESIAN_POINT ( 'NONE',  ( 21.80757117620698438, -274.3975131968944652, -221.1585712227553415 ) ) ;
#61694=CARTESIAN_POINT ( 'NONE',  ( -90.53302526049461108, -295.7618794506587392, -219.2842815334317379 ) ) ;
#61695=CARTESIAN_POINT ( 'NONE',  ( 16.50995796980268793, -278.1368192719580748, -321.4577362698927914 ) ) ;
#61696=CARTESIAN_POINT ( 'NONE',  ( -5.986066114848981101, -272.6083415682933833, -203.0730083407317750 ) ) ;
#61697=CARTESIAN_POINT ( 'NONE',  ( -107.2427461482248390, -297.4600600140454958, -292.9079945410235837 ) ) ;
#61698=CARTESIAN_POINT ( 'NONE',  ( -109.1849137494126580, -297.4393913849345381, -285.0105136649997917 ) ) ;
#61700=CARTESIAN_POINT ( 'NONE',  ( -100.1034411153165991, -298.7290044283499810, -227.1247058303513882 ) ) ;
#61701=CARTESIAN_POINT ( 'NONE',  ( -32.04458707427265551, -296.1181581694353326, -195.1962435526542379 ) ) ;
#61702=CARTESIAN_POINT ( 'NONE',  ( 31.89490615158765152, -293.8904685894862041, -246.7475723268689194 ) ) ;
#61703=CARTESIAN_POINT ( 'NONE',  ( 19.81483159065459176, -291.4761587397313178, -223.9892042655206126 ) ) ;
#61705=CARTESIAN_POINT ( 'NONE',  ( 2.380857498295728458, -275.0618641025213833, -204.4699553064321549 ) ) ;
#61706=CARTESIAN_POINT ( 'NONE',  ( -78.85681564543277489, -273.6421770151165447, -210.2539385205406575 ) ) ;
#61707=CARTESIAN_POINT ( 'NONE',  ( 35.60603866203060619, -283.7736923825752342, -289.2564669135535951 ) ) ;
#61708=CARTESIAN_POINT ( 'NONE',  ( 1.827186276290179823, -281.2244271097814590, -336.0809522062260726 ) ) ;
#61709=CARTESIAN_POINT ( 'NONE',  ( -104.8900091063205480, -277.4245540456624326, -307.1107947223466113 ) ) ;
#61711=CARTESIAN_POINT ( 'NONE',  ( -110.3887706229250085, -283.8140340680066629, -265.4441880852010058 ) ) ;
#61712=CARTESIAN_POINT ( 'NONE',  ( 22.77319316338241606, -280.1672660011499829, -315.4857014618617086 ) ) ;
#61713=CARTESIAN_POINT ( 'NONE',  ( -11.06042472033237800, -275.2774481595370730, -339.0973491870378211 ) ) ;
#61714=CARTESIAN_POINT ( 'NONE',  ( -103.2298473196971713, -281.0295542470021246, -234.4242296509845858 ) ) ;
#61717=CARTESIAN_POINT ( 'NONE',  ( -36.92344601342082910, -272.4572174972324206, -194.1493462586157079 ) ) ;
#61719=CARTESIAN_POINT ( 'NONE',  ( -73.19930813355162513, -279.5265209579058023, -336.4383094284160620 ) ) ;
#61722=CARTESIAN_POINT ( 'NONE',  ( -73.56376682094546027, -285.4486933774028898, -336.7314492666141632 ) ) ;
#61724=CARTESIAN_POINT ( 'NONE',  ( -4.661502229877561909, -286.6216043090495305, -337.8806908614707822 ) ) ;
#61726=CARTESIAN_POINT ( 'NONE',  ( -110.6077436098145768, -295.4045861318891752, -265.9773551691940270 ) ) ;
#61727=CARTESIAN_POINT ( 'NONE',  ( -5.280047729139999646, -286.7652392031147883, -337.3156990769847425 ) ) ;
#61728=CARTESIAN_POINT ( 'NONE',  ( -113.2098679957031493, -271.2709011634024137, -296.4525692007673570 ) ) ;
#61729=CARTESIAN_POINT ( 'NONE',  ( -112.2072278674401531, -294.6096294047426909, -265.8718638674570798 ) ) ;
#61730=CARTESIAN_POINT ( 'NONE',  ( -70.74509997123259097, -284.0994285422036114, -201.7541166295424375 ) ) ;
#61731=CARTESIAN_POINT ( 'NONE',  ( 32.99997958420892274, -283.4470534781863762, -292.8545588516321345 ) ) ;
#61732=CARTESIAN_POINT ( 'NONE',  ( -96.39918681714449633, -282.1420044092341186, -318.1956631655522187 ) ) ;
#61733=CARTESIAN_POINT ( 'NONE',  ( 5.844624518468904739, -288.4484808899330801, -329.2793726299055947 ) ) ;
#61734=CARTESIAN_POINT ( 'NONE',  ( -72.42648506604072622, -281.0033995892246139, -205.6739261749698642 ) ) ;
#61735=CARTESIAN_POINT ( 'NONE',  ( 29.11508965688805617, -281.9416790250525651, -239.6440461672289644 ) ) ;
#61736=CARTESIAN_POINT ( 'NONE',  ( 30.22406979101944557, -289.9715057260395952, -303.8446337056924449 ) ) ;
#61738=CARTESIAN_POINT ( 'NONE',  ( -96.93607219985013046, -273.2069953152112021, -221.5808175174131236 ) ) ;
#61739=CARTESIAN_POINT ( 'NONE',  ( -108.5128722171562714, -292.2382798057213336, -293.0376917566769635 ) ) ;
#61741=CARTESIAN_POINT ( 'NONE',  ( -115.3288506153726871, -298.8376638359844719, -288.1938231032136741 ) ) ;
#61743=CARTESIAN_POINT ( 'NONE',  ( 35.85559431217997428, -273.3323524544736642, -253.2116385803447258 ) ) ;
#61745=CARTESIAN_POINT ( 'NONE',  ( -55.89541940631961836, -293.6870707472124309, -344.2678153406051251 ) ) ;
#61746=CARTESIAN_POINT ( 'NONE',  ( -38.07507084467897585, -273.3913078115546114, -197.2628633115357673 ) ) ;
#61747=CARTESIAN_POINT ( 'NONE',  ( 28.85900960654986847, -289.5066803082945057, -302.7366300421691676 ) ) ;
#61748=CARTESIAN_POINT ( 'NONE',  ( -65.68328017059339174, -285.1880983808048882, -338.7468920703397544 ) ) ;
#61749=CARTESIAN_POINT ( 'NONE',  ( -39.21557508759703126, -293.4543665593869832, -193.9603899851933875 ) ) ;
#61750=CARTESIAN_POINT ( 'NONE',  ( -109.9681002367401135, -292.1739520399975163, -246.1389439068909439 ) ) ;
#61751=CARTESIAN_POINT ( 'NONE',  ( -52.36769633436161797, -291.6877866536235047, -198.8723961294197125 ) ) ;
#61752=CARTESIAN_POINT ( 'NONE',  ( -104.0280200930546641, -287.0064152868697533, -236.0400548394829627 ) ) ;
#61753=CARTESIAN_POINT ( 'NONE',  ( -2.392038180182951113, -280.6683031818170662, -201.7350128943758705 ) ) ;
#61754=CARTESIAN_POINT ( 'NONE',  ( -111.1878491669540381, -294.8366627391303609, -254.2989303348274177 ) ) ;
#61755=CARTESIAN_POINT ( 'NONE',  ( -13.42395082226543224, -282.5832479676305979, -343.5522463564098530 ) ) ;
#61756=CARTESIAN_POINT ( 'NONE',  ( 12.35616036713719268, -276.6128957670105706, -215.1467677941314491 ) ) ;
#61757=CARTESIAN_POINT ( 'NONE',  ( -21.39648532958013050, -288.7662352645559167, -200.3538533559491555 ) ) ;
#61758=CARTESIAN_POINT ( 'NONE',  ( -88.39750893331228099, -275.8983340109349456, -326.3397734286518244 ) ) ;
#61760=CARTESIAN_POINT ( 'NONE',  ( -61.56103168232197476, -282.8829826070968920, -339.3448907544527628 ) ) ;
#61761=CARTESIAN_POINT ( 'NONE',  ( -105.8275000105147257, -280.2022760054974810, -235.9252415360201098 ) ) ;
#61762=CARTESIAN_POINT ( 'NONE',  ( 23.09477475923405265, -287.2457204057055264, -317.7135876576458031 ) ) ;
#61763=CARTESIAN_POINT ( 'NONE',  ( -14.55543027648865007, -294.1117480074439641, -199.9426550750086733 ) ) ;
#61764=CARTESIAN_POINT ( 'NONE',  ( 11.25960873806925200, -276.3123692145800305, -211.6039555493101432 ) ) ;
#61765=CARTESIAN_POINT ( 'NONE',  ( 25.72848013901437980, -276.2918157665897638, -227.0314313166890656 ) ) ;
#61766=CARTESIAN_POINT ( 'NONE',  ( -110.1584954130612601, -278.4536533850556452, -265.1925273706037842 ) ) ;
#61767=CARTESIAN_POINT ( 'NONE',  ( -47.54736812926478251, -299.9224262400600765, -196.1744654553654925 ) ) ;
#61768=CARTESIAN_POINT ( 'NONE',  ( -88.94065543887441549, -283.3248562392004146, -216.1617062192939613 ) ) ;
#61769=CARTESIAN_POINT ( 'NONE',  ( -4.609280072800064687, -292.1384201422026194, -200.6880746373742852 ) ) ;
#61770=CARTESIAN_POINT ( 'NONE',  ( 26.78272143995865662, -289.6990484588970389, -311.6227404202854814 ) ) ;
#61771=CARTESIAN_POINT ( 'NONE',  ( -25.34502083228317204, -291.1288499121718019, -197.9885670057450398 ) ) ;
#61773=CARTESIAN_POINT ( 'NONE',  ( -44.82116619460498441, -290.5341019360635073, -194.2647721673558578 ) ) ;
#61774=CARTESIAN_POINT ( 'NONE',  ( 20.20217807723913950, -292.5851971834346159, -225.3876807377890543 ) ) ;
#61776=CARTESIAN_POINT ( 'NONE',  ( -82.65887779399071178, -290.7351921953559781, -332.2307059666654254 ) ) ;
#61777=CARTESIAN_POINT ( 'NONE',  ( -110.3010914625495928, -278.8458396717747405, -273.3635674477395696 ) ) ;
#61778=CARTESIAN_POINT ( 'NONE',  ( -111.2975919183238460, -295.2171995835493021, -290.6593587899989757 ) ) ;
#61779=CARTESIAN_POINT ( 'NONE',  ( -78.47495036605826613, -286.1652749493692909, -205.3890585162750426 ) ) ;
#61780=CARTESIAN_POINT ( 'NONE',  ( -30.88985682315427894, -286.4648368923487851, -193.6398219820470388 ) ) ;
#61782=CARTESIAN_POINT ( 'NONE',  ( -108.9994259045149931, -284.7002132494902185, -284.4059684052884336 ) ) ;
#61783=CARTESIAN_POINT ( 'NONE',  ( -113.9563424175841249, -273.7439901500910651, -270.3762929349610431 ) ) ;
#61784=CARTESIAN_POINT ( 'NONE',  ( 137.3882156427991390, 180.6064192809313909, -240.3616213788371283 ) ) ;
#61785=CARTESIAN_POINT ( 'NONE',  ( 178.9112196240999992, 251.4731691113353236, -164.2126119813759715 ) ) ;
#61786=CARTESIAN_POINT ( 'NONE',  ( 3.027542779753411573, -273.8063717156109647, -209.2847822823411263 ) ) ;
#61787=CARTESIAN_POINT ( 'NONE',  ( 35.95223312036172558, -274.4528782497610564, -268.8693332707915147 ) ) ;
#61788=CARTESIAN_POINT ( 'NONE',  ( -85.17325803495880621, -296.9191686114214690, -210.0977877455485157 ) ) ;
#61789=CARTESIAN_POINT ( 'NONE',  ( -92.77482839370959766, -239.7623855883933857, -339.1558859853604986 ) ) ;
#61790=CARTESIAN_POINT ( 'NONE',  ( 27.22359873830451704, -274.7795192335319712, -311.5036896027992839 ) ) ;
#61791=CARTESIAN_POINT ( 'NONE',  ( -67.49052412720305938, -275.4113190183768438, -202.7526883425835251 ) ) ;
#61793=CARTESIAN_POINT ( 'NONE',  ( -105.3412525188624045, -274.0924095737876769, -234.7843024903218065 ) ) ;
#61794=CARTESIAN_POINT ( 'NONE',  ( -58.70113780472167520, -289.8281797772984874, -340.2835781494169396 ) ) ;
#61795=CARTESIAN_POINT ( 'NONE',  ( -71.99204873566625906, -296.3014567289501429, -338.9432742808064631 ) ) ;
#61796=CARTESIAN_POINT ( 'NONE',  ( -68.15857400180846071, -298.1506699728736862, -199.8072200716321731 ) ) ;
#61797=CARTESIAN_POINT ( 'NONE',  ( -92.18927209325447336, -296.0311434916832241, -318.5352173933906670 ) ) ;
#61800=CARTESIAN_POINT ( 'NONE',  ( -48.26125739924071212, -279.1100843173926478, -345.1808229464237456 ) ) ;
#61802=CARTESIAN_POINT ( 'NONE',  ( 27.80259150927189182, -280.5222561422730791, -229.3253587791473080 ) ) ;
#61803=CARTESIAN_POINT ( 'NONE',  ( -36.45132540264958010, -277.9820129269591575, -343.6035076930010064 ) ) ;
#61804=CARTESIAN_POINT ( 'NONE',  ( -25.90013305583154946, -278.6684842869273666, -345.4814518129636554 ) ) ;
#61805=CARTESIAN_POINT ( 'NONE',  ( -103.5428822824225534, -276.0962889277454337, -306.3584829065293889 ) ) ;
#61806=CARTESIAN_POINT ( 'NONE',  ( -109.6445916786506274, -273.1874762735358217, -259.5137285536690683 ) ) ;
#61807=CARTESIAN_POINT ( 'NONE',  ( 9.416850655049715968, -297.2234503871736706, -196.7834957107979790 ) ) ;
#61809=CARTESIAN_POINT ( 'NONE',  ( -109.2857212142774301, -278.5546557279030822, -282.8066459144263263 ) ) ;
#61810=CARTESIAN_POINT ( 'NONE',  ( 36.66311010202157661, -286.4814646207431679, -289.7669505293973771 ) ) ;
#61811=CARTESIAN_POINT ( 'NONE',  ( 10.49007060466537666, -276.7123369542541695, -212.5258196686554015 ) ) ;
#61813=CARTESIAN_POINT ( 'NONE',  ( -106.1879713544767299, -289.4203594134405080, -295.1157673435341735 ) ) ;
#61814=CARTESIAN_POINT ( 'NONE',  ( -97.96918328365069328, -283.2678753185803089, -317.6646175712123750 ) ) ;
#61816=CARTESIAN_POINT ( 'NONE',  ( 31.26557468018033248, -280.1587699166595371, -298.1282902344638615 ) ) ;
#61818=CARTESIAN_POINT ( 'NONE',  ( 9.666770678202762923, -279.2881889945341527, -213.6768483925877433 ) ) ;
#61819=CARTESIAN_POINT ( 'NONE',  ( -98.52584599908749396, -283.2116020439131034, -227.9379539621903916 ) ) ;
#61820=CARTESIAN_POINT ( 'NONE',  ( -13.52940195129821177, -290.7433003103289479, -341.5342403475561923 ) ) ;
#61821=CARTESIAN_POINT ( 'NONE',  ( -109.8821778902806727, -279.6105375055316244, -281.5418867918415913 ) ) ;
#61823=CARTESIAN_POINT ( 'NONE',  ( -14.50043690629413362, -294.3482656844052485, -198.8693767043140213 ) ) ;
#61824=CARTESIAN_POINT ( 'NONE',  ( -111.7209650602492985, -276.9898321192069943, -254.7517902831631886 ) ) ;
#61825=CARTESIAN_POINT ( 'NONE',  ( -8.691091834693455809, -277.3185046426877420, -337.6281954159796328 ) ) ;
#61826=CARTESIAN_POINT ( 'NONE',  ( -96.58339680265815730, -285.9190198425260405, -316.6261134549433223 ) ) ;
#61827=DIRECTION ( 'NONE',  ( -1.000000000000000000, -0.000000000000000000, -0.000000000000000000 ) ) ;
#61828=CARTESIAN_POINT ( 'NONE',  ( -111.7115557554895133, -292.3011281923740512, -283.7921675866518854 ) ) ;
#61829=CARTESIAN_POINT ( 'NONE',  ( -78.64588175427462602, -293.6078344819043764, -333.0237903765516307 ) ) ;
#61830=CARTESIAN_POINT ( 'NONE',  ( 37.86756833272411882, -286.5512697743581043, -254.5580960424597663 ) ) ;
#61831=CARTESIAN_POINT ( 'NONE',  ( -106.4527194294426380, -289.2953449765810774, -244.3297865404355491 ) ) ;
#61833=CARTESIAN_POINT ( 'NONE',  ( 28.46466553028474777, -274.6790778534708011, -303.1983470878130333 ) ) ;
#61834=CARTESIAN_POINT ( 'NONE',  ( -15.24741628013194905, -292.9027502300475021, -341.2862498786924448 ) ) ;
#61837=CARTESIAN_POINT ( 'NONE',  ( -79.19778501283552430, -289.9787171685997009, -206.4953334003015186 ) ) ;
#61838=CARTESIAN_POINT ( 'NONE',  ( -70.35842355555413974, -287.2096857055699388, -204.3444710870405459 ) ) ;
#61839=CARTESIAN_POINT ( 'NONE',  ( -4.787788183634853034, -286.8691795759041838, -339.0355591239228943 ) ) ;
#61841=CARTESIAN_POINT ( 'NONE',  ( -98.60760005059161415, -286.5387798743906842, -229.5951465862859777 ) ) ;
#61843=CARTESIAN_POINT ( 'NONE',  ( -81.58433094222112913, -286.2350274175871618, -212.0928474995660338 ) ) ;
#61844=CARTESIAN_POINT ( 'NONE',  ( 20.04119715018747883, -294.8589025322291377, -221.4987077065173082 ) ) ;
#61846=CARTESIAN_POINT ( 'NONE',  ( -112.9366163918105883, -276.6526533676092185, -268.7402689221095216 ) ) ;
#61847=CARTESIAN_POINT ( 'NONE',  ( -6.579250699816183712, -276.9924331444652239, -340.9403477577145054 ) ) ;
#61848=CARTESIAN_POINT ( 'NONE',  ( 19.31545630746252584, -290.9419942586628736, -220.3487549054204919 ) ) ;
#61849=CARTESIAN_POINT ( 'NONE',  ( -91.05816846703244494, -279.3148217051064535, -215.1184886317592486 ) ) ;
#61850=CARTESIAN_POINT ( 'NONE',  ( -110.4916491207447251, -298.3394665757891175, -285.2884422388504504 ) ) ;
#61853=CARTESIAN_POINT ( 'NONE',  ( -108.4027662223042370, -276.9713366982268781, -248.8857747593772558 ) ) ;
#61854=CARTESIAN_POINT ( 'NONE',  ( 28.00644727378776366, -280.0435018214005254, -307.2720657957934236 ) ) ;
#61856=CARTESIAN_POINT ( 'NONE',  ( 38.86316984842187594, -273.9707267780482880, -265.5033829570034527 ) ) ;
#61857=CARTESIAN_POINT ( 'NONE',  ( -84.91102871554552678, -297.2420197399135304, -326.7119077935265068 ) ) ;
#61858=CARTESIAN_POINT ( 'NONE',  ( 35.31180129020641800, -280.7848916590746171, -295.0813327202610594 ) ) ;
#61859=CARTESIAN_POINT ( 'NONE',  ( 10.45411433616792252, -295.3141056561549931, -325.8495723414083045 ) ) ;
#61860=CARTESIAN_POINT ( 'NONE',  ( -60.01800384170071823, -299.0795797461608458, -197.2369145107730901 ) ) ;
#61861=CARTESIAN_POINT ( 'NONE',  ( -85.32086176758463125, -273.0344852712404986, -215.2474979412859284 ) ) ;
#61862=CARTESIAN_POINT ( 'NONE',  ( -99.98365724561688239, -293.1101111241162016, -229.0237257701417661 ) ) ;
#61863=CARTESIAN_POINT ( 'NONE',  ( 18.35003018030980826, -286.9910099010896261, -217.1106295021070025 ) ) ;
#61864=CARTESIAN_POINT ( 'NONE',  ( 38.32231115665356924, -273.6304875881065186, -265.5423339125887878 ) ) ;
#61865=CARTESIAN_POINT ( 'NONE',  ( -31.82889751765750219, -288.8178525183249690, -347.2160763128621284 ) ) ;
#61866=CARTESIAN_POINT ( 'NONE',  ( 1.426009652876563782, -287.5788774304659228, -332.4938237524259534 ) ) ;
#61867=CARTESIAN_POINT ( 'NONE',  ( -102.8503788927215084, -289.0380696716037505, -233.8424425862099554 ) ) ;
#61870=CARTESIAN_POINT ( 'NONE',  ( 31.45524049038889203, -287.3870214156676752, -294.9572437573685875 ) ) ;
#61872=CARTESIAN_POINT ( 'NONE',  ( -81.41662811903604791, -284.5764467986614363, -333.2765623931563823 ) ) ;
#61873=CARTESIAN_POINT ( 'NONE',  ( 38.58205543801906146, -292.7530540957635594, -281.6926471693149097 ) ) ;
#61874=CARTESIAN_POINT ( 'NONE',  ( -22.73965536964717415, -281.8360094825371789, -195.5195905845205573 ) ) ;
#61875=CARTESIAN_POINT ( 'NONE',  ( -41.00166701588969431, -281.3221999881022839, -193.9287495705772812 ) ) ;
#61876=CARTESIAN_POINT ( 'NONE',  ( -7.255417066997774889, -282.4795289046936659, -336.8866015445254334 ) ) ;
#61877=CARTESIAN_POINT ( 'NONE',  ( -46.11751120001068216, -279.1634940181720594, -344.8979323227834470 ) ) ;
#61878=CARTESIAN_POINT ( 'NONE',  ( -105.9577023256337185, -296.1008837772716333, -305.4191531795616470 ) ) ;
#61879=CARTESIAN_POINT ( 'NONE',  ( -27.23884825033445978, -275.4982778080797630, -197.5144380451885979 ) ) ;
#61880=CARTESIAN_POINT ( 'NONE',  ( -110.8931712491901749, -288.7402756840113511, -257.3375499817615832 ) ) ;
#61881=CARTESIAN_POINT ( 'NONE',  ( -70.59552866683937111, -296.5233027525680995, -205.0140867333433334 ) ) ;
#61884=CARTESIAN_POINT ( 'NONE',  ( -99.31927630328665657, -287.0335818043434983, -229.1289188010974271 ) ) ;
#61885=CARTESIAN_POINT ( 'NONE',  ( -39.08696827218560799, -296.1532395277390606, -347.0321460828203612 ) ) ;
#61886=CARTESIAN_POINT ( 'NONE',  ( -105.6631424160158161, -285.5502410245010765, -244.3597104883670283 ) ) ;
#61887=CARTESIAN_POINT ( 'NONE',  ( 18.72315065344179885, -275.3282999676742406, -322.7972955681944427 ) ) ;
#61888=CARTESIAN_POINT ( 'NONE',  ( -112.5420391258298878, -291.4055387729696918, -254.2296795115352381 ) ) ;
#61889=CARTESIAN_POINT ( 'NONE',  ( -32.36353232082194609, -284.2538528623061325, -194.7470828097350477 ) ) ;
#61890=CARTESIAN_POINT ( 'NONE',  ( 15.42058298479754974, -293.1065686548539020, -214.2354055956243428 ) ) ;
#61891=CARTESIAN_POINT ( 'NONE',  ( -102.8625357173389716, -290.4487604618014416, -302.5963097822548207 ) ) ;
#61892=CARTESIAN_POINT ( 'NONE',  ( 128.9467878515196162, -299.5541904835127980, -195.3611179825600175 ) ) ;
#61894=CARTESIAN_POINT ( 'NONE',  ( -107.2659097474429899, -264.6957166766804903, -305.4471583230359784 ) ) ;
#61895=CARTESIAN_POINT ( 'NONE',  ( -47.14791445113996105, -284.6947006952134984, -346.0350627207626530 ) ) ;
#61896=CARTESIAN_POINT ( 'NONE',  ( -69.91165696735023971, -286.9809262143061801, -337.9199732462171255 ) ) ;
#61898=CARTESIAN_POINT ( 'NONE',  ( 30.31202254033113164, -280.0953339040042920, -242.1263896873278441 ) ) ;
#61899=CARTESIAN_POINT ( 'NONE',  ( 31.83441851047345850, -275.6539562771033616, -304.2524577740957170 ) ) ;
#61900=CARTESIAN_POINT ( 'NONE',  ( -110.0774823086269265, -280.7787490018314998, -252.7675276394120090 ) ) ;
#61901=CARTESIAN_POINT ( 'NONE',  ( 104.9614017666556407, 114.4850001852085768, -281.3012701160373581 ) ) ;
#61902=CARTESIAN_POINT ( 'NONE',  ( 34.03061303885380084, -280.4750190945214854, -297.6484631254596138 ) ) ;
#61903=CARTESIAN_POINT ( 'NONE',  ( -110.8074603620060259, -282.7436680862338108, -257.0746221734004280 ) ) ;
#61904=CARTESIAN_POINT ( 'NONE',  ( -36.22580109295046924, -299.8260745248370540, -194.3741156519464823 ) ) ;
#61905=CARTESIAN_POINT ( 'NONE',  ( -28.88263444934930391, -295.4345110711901157, -342.9823661880266741 ) ) ;
#61907=CARTESIAN_POINT ( 'NONE',  ( -28.02735765637791587, -290.8575379229812370, -197.4095014941110549 ) ) ;
#61908=CARTESIAN_POINT ( 'NONE',  ( 39.03735201124917609, -276.3208549875936342, -279.7272370890412958 ) ) ;
#61909=CARTESIAN_POINT ( 'NONE',  ( 29.08604667910517705, -275.1425530550601479, -239.9674884841780624 ) ) ;
#61910=CARTESIAN_POINT ( 'NONE',  ( 7.067237077276159241, -273.5612970577896590, -207.7712323599128865 ) ) ;
#61911=CARTESIAN_POINT ( 'NONE',  ( -32.12788024951596100, -272.1177395468341729, -195.5298027718906724 ) ) ;
#61915=CARTESIAN_POINT ( 'NONE',  ( -37.52755671434548645, -284.1342414025808694, -343.6824772921255544 ) ) ;
#61916=CARTESIAN_POINT ( 'NONE',  ( 19.04679684927533856, -284.0137909534382743, -321.3725098920343157 ) ) ;
#61917=CARTESIAN_POINT ( 'NONE',  ( -87.75881478372605216, -284.6733862353213453, -217.4271287337541310 ) ) ;
#61918=CARTESIAN_POINT ( 'NONE',  ( -41.92642186165905116, -275.5107209694161838, -344.0313078368051265 ) ) ;
#61919=CARTESIAN_POINT ( 'NONE',  ( -26.54002244950858724, -284.7738365682291715, -343.8584321605129617 ) ) ;
#61920=CARTESIAN_POINT ( 'NONE',  ( -110.8615457380539340, -276.9568481582520008, -276.1139129462578694 ) ) ;
#61922=CARTESIAN_POINT ( 'NONE',  ( 28.13121531422804011, -276.1861268284859534, -237.3834980543300617 ) ) ;
#61924=CARTESIAN_POINT ( 'NONE',  ( -112.2466121693338295, -279.5696559271012802, -253.2318163756536649 ) ) ;
#61927=CARTESIAN_POINT ( 'NONE',  ( -37.99593755795142869, -287.9044470443560044, -194.5991390091889457 ) ) ;
#61928=CARTESIAN_POINT ( 'NONE',  ( -86.60623650512609117, -294.9552560944425750, -324.4500002238842740 ) ) ;
#61929=CARTESIAN_POINT ( 'NONE',  ( -114.0855863780710564, -289.9616909165201832, -265.4940131380938624 ) ) ;
#61930=EDGE_CURVE ( 'NONE', #85436, #58191, #12352, .T. ) ;
#61931=CARTESIAN_POINT ( 'NONE',  ( 25.82709335916489835, -285.2678952497789737, -231.7906948365903474 ) ) ;
#61932=CARTESIAN_POINT ( 'NONE',  ( 35.70694275621561786, -286.2433843592186236, -279.2645268563812238 ) ) ;
#61933=CARTESIAN_POINT ( 'NONE',  ( -69.43702529255786260, -289.8638040297339558, -203.6548155200333099 ) ) ;
#61934=CARTESIAN_POINT ( 'NONE',  ( -101.3450524992450283, -286.2473712684401903, -234.3305891629819655 ) ) ;
#61935=CARTESIAN_POINT ( 'NONE',  ( -34.39582984381018349, -275.0149512536929137, -345.3032456508428254 ) ) ;
#61936=CARTESIAN_POINT ( 'NONE',  ( -29.52453639315038103, -284.5494708129585888, -194.5631472584524886 ) ) ;
#61937=CARTESIAN_POINT ( 'NONE',  ( -97.50377935892751680, -299.1640323899787859, -225.5565875564690543 ) ) ;
#61938=CARTESIAN_POINT ( 'NONE',  ( 36.75407569789460638, -285.3890465478248757, -257.6422897795365543 ) ) ;
#61939=CARTESIAN_POINT ( 'NONE',  ( 34.56297956985122966, -282.3098040861296454, -256.3981476393850585 ) ) ;
#61940=CARTESIAN_POINT ( 'NONE',  ( -15.46098991042042492, -290.7698964495539826, -342.3270414939656803 ) ) ;
#61943=CARTESIAN_POINT ( 'NONE',  ( -103.3331209589990038, -297.9848315658342699, -307.2708249365308006 ) ) ;
#61944=CARTESIAN_POINT ( 'NONE',  ( -49.44011554625806326, -277.8977340686983553, -196.3433566639332071 ) ) ;
#61945=CARTESIAN_POINT ( 'NONE',  ( -16.66022970355939847, -291.5099242788823517, -196.3581747903004100 ) ) ;
#61946=CARTESIAN_POINT ( 'NONE',  ( -108.2221050657300765, -295.2209196503710587, -249.8085363459832422 ) ) ;
#61947=CARTESIAN_POINT ( 'NONE',  ( 27.28077401663080792, -280.7113718197099388, -305.3636794913035146 ) ) ;
#61948=CARTESIAN_POINT ( 'NONE',  ( 16.50500617276932402, -272.9042914306951388, -218.8875793137998471 ) ) ;
#61949=CARTESIAN_POINT ( 'NONE',  ( 33.78125297579861552, -294.6245412795799439, -251.8470957023897085 ) ) ;
#61950=CARTESIAN_POINT ( 'NONE',  ( 39.58706461736020543, -290.0519495502702512, -270.3284710469133074 ) ) ;
#61951=CARTESIAN_POINT ( 'NONE',  ( -103.2411790222717087, -295.5383631549463530, -231.7866989438958569 ) ) ;
#61952=CARTESIAN_POINT ( 'NONE',  ( 18.76610242438108500, -292.4987351209083499, -321.6811558648663549 ) ) ;
#61954=CARTESIAN_POINT ( 'NONE',  ( -92.12384150760014734, -292.6751418966863412, -221.2068201637980280 ) ) ;
#61957=CARTESIAN_POINT ( 'NONE',  ( -38.91127114659439457, -292.8347961503388319, -197.2164792571050214 ) ) ;
#61959=CARTESIAN_POINT ( 'NONE',  ( -91.27452030472841216, -281.8346503915630024, -322.9886555450844412 ) ) ;
#61960=CARTESIAN_POINT ( 'NONE',  ( -7.270246031502023421, -292.4579246911467862, -203.8426419889135843 ) ) ;
#61961=CARTESIAN_POINT ( 'NONE',  ( 21.61001375088902776, -282.2191246445926822, -319.8959080874147389 ) ) ;
#61962=CARTESIAN_POINT ( 'NONE',  ( -33.06416573163687644, -282.6664083488201982, -347.2341673600084277 ) ) ;
#61963=CARTESIAN_POINT ( 'NONE',  ( 9.098239688096295907, -286.4127103745565819, -329.0412714693239877 ) ) ;
#61964=CARTESIAN_POINT ( 'NONE',  ( 32.91988840049522480, -280.4158573086644992, -300.2620116619760324 ) ) ;
#61965=CARTESIAN_POINT ( 'NONE',  ( 39.03834907244375785, -286.5590980742975376, -277.2589867325837076 ) ) ;
#61967=CARTESIAN_POINT ( 'NONE',  ( 33.11658072861089153, -295.4400758530240978, -292.3172349924735727 ) ) ;
#61968=CARTESIAN_POINT ( 'NONE',  ( 33.64365787055034929, -277.3405534871892542, -298.7825623721442980 ) ) ;
#61969=CARTESIAN_POINT ( 'NONE',  ( -39.69766389053298639, -279.6885039081295190, -197.3654668857656418 ) ) ;
#61970=CARTESIAN_POINT ( 'NONE',  ( 39.44090743966724233, -293.6465202733311344, -264.5791477658112854 ) ) ;
#61971=CARTESIAN_POINT ( 'NONE',  ( -1.088236823255665175, -280.6548145239515293, -336.6705762207873818 ) ) ;
#61974=CARTESIAN_POINT ( 'NONE',  ( 35.65801755045901444, -292.6880730879821044, -276.2305018100163920 ) ) ;
#61975=CARTESIAN_POINT ( 'NONE',  ( -94.04192548860704903, -295.2335761265449605, -221.1910238512157036 ) ) ;
#61977=CARTESIAN_POINT ( 'NONE',  ( -4.314445822074130632, -294.1122834535618153, -335.5455879334134579 ) ) ;
#61980=CARTESIAN_POINT ( 'NONE',  ( 30.91033621190086578, -290.8380690714489560, -254.8156830097664738 ) ) ;
#61981=CARTESIAN_POINT ( 'NONE',  ( -36.53163284054154758, -297.1208148081067861, -193.5965360629227803 ) ) ;
#61982=CARTESIAN_POINT ( 'NONE',  ( 25.68106271542059105, -280.2543228823050754, -312.4139043813443664 ) ) ;
#61983=CARTESIAN_POINT ( 'NONE',  ( -85.21742987243534628, -286.7216552534935090, -210.6852202275717900 ) ) ;
#61984=CARTESIAN_POINT ( 'NONE',  ( -26.47698553936530530, -288.7435041215287583, -342.5991326974644835 ) ) ;
#61985=CARTESIAN_POINT ( 'NONE',  ( -45.97024486336496096, -278.6835328600971025, -343.5986705769190053 ) ) ;
#61986=CARTESIAN_POINT ( 'NONE',  ( -108.2617752005481151, -294.8764038408161241, -246.9124571777710173 ) ) ;
#61987=CARTESIAN_POINT ( 'NONE',  ( -107.9680292408225597, -274.4347567752539021, -248.7765098765487437 ) ) ;
#61988=CARTESIAN_POINT ( 'NONE',  ( -109.6800331247346350, -277.1831215343365216, -282.8570925155178202 ) ) ;
#61990=CARTESIAN_POINT ( 'NONE',  ( -112.4428150783791551, -272.5980163036712156, -253.3663382617036177 ) ) ;
#61991=CARTESIAN_POINT ( 'NONE',  ( -111.5562268422951888, -292.3893012345352531, -276.7779036592502848 ) ) ;
#61992=CARTESIAN_POINT ( 'NONE',  ( 37.57452534993619508, -295.3291901494370677, -284.3600939016120606 ) ) ;
#61994=CARTESIAN_POINT ( 'NONE',  ( -94.17831061124951475, -290.5542076525889570, -316.3338531345516458 ) ) ;
#61997=CARTESIAN_POINT ( 'NONE',  ( -113.5504586543767545, -297.0700329378709057, -281.0239587129651113 ) ) ;
#61998=CARTESIAN_POINT ( 'NONE',  ( -99.67802396944000520, -288.1137912945842459, -313.4248871045240890 ) ) ;
#61999=CARTESIAN_POINT ( 'NONE',  ( -54.59455488739089191, -298.1695626392007625, -195.3405655046613845 ) ) ;
#62002=CARTESIAN_POINT ( 'NONE',  ( -103.1902414082874770, -291.5646672956302154, -309.0230412759524370 ) ) ;
#62003=CARTESIAN_POINT ( 'NONE',  ( 13.84574458161073096, -290.9090924074130839, -334.4957818155094174 ) ) ;
#62004=CARTESIAN_POINT ( 'NONE',  ( -105.7799410536550226, -286.1549196048806607, -300.6305018968373588 ) ) ;
#62005=CARTESIAN_POINT ( 'NONE',  ( 34.51213430789309911, -286.4594353561856792, -296.5078931113799285 ) ) ;
#62006=CARTESIAN_POINT ( 'NONE',  ( -2.026527581831383706, -272.5208028060419565, -204.3848569729614439 ) ) ;
#62007=CARTESIAN_POINT ( 'NONE',  ( -103.3178379009176666, -274.9336751837110455, -235.7753055979397345 ) ) ;
#62008=CARTESIAN_POINT ( 'NONE',  ( -104.1483268116819971, -288.1956878634434247, -303.1969037359135086 ) ) ;
#62009=CARTESIAN_POINT ( 'NONE',  ( -37.10662138636033802, -278.9096130583695867, -346.1384066330168139 ) ) ;
#62011=CARTESIAN_POINT ( 'NONE',  ( -37.00832681121497103, -280.0564418895975223, -197.3618792041206689 ) ) ;
#62012=CARTESIAN_POINT ( 'NONE',  ( 15.33858816733796360, -280.1692949061843478, -219.6066496645920836 ) ) ;
#62013=CARTESIAN_POINT ( 'NONE',  ( 39.31510157568975927, -276.6777088617315030, -274.0154680389487680 ) ) ;
#62014=CARTESIAN_POINT ( 'NONE',  ( 37.29412289443150286, -280.1295961886257828, -253.0551699148767568 ) ) ;
#62015=CARTESIAN_POINT ( 'NONE',  ( -113.1081836994901408, -270.5045731412160990, -283.7362657651427185 ) ) ;
#62016=CARTESIAN_POINT ( 'NONE',  ( 31.64909690800963560, -276.9282843539091346, -304.1436361792107164 ) ) ;
#62018=CARTESIAN_POINT ( 'NONE',  ( -76.09742436145226918, -275.0647115253971720, -204.5680114361689732 ) ) ;
#62019=CARTESIAN_POINT ( 'NONE',  ( 21.27581636871892101, -295.4090924074130839, -223.5744983911110353 ) ) ;
#62023=CARTESIAN_POINT ( 'NONE',  ( 18.00054895498326957, -287.9492933628943661, -222.2834564266263442 ) ) ;
#62024=CARTESIAN_POINT ( 'NONE',  ( 37.96794746350486349, -289.1840281974967297, -260.2402982059978171 ) ) ;
#62025=CARTESIAN_POINT ( 'NONE',  ( -53.43903441008619382, -288.6127324944325778, -341.6686806729079535 ) ) ;
#62026=CARTESIAN_POINT ( 'NONE',  ( -46.49195521434227629, -285.4466288686685402, -193.9687117173135107 ) ) ;
#62028=CARTESIAN_POINT ( 'NONE',  ( 32.10050812918746743, -280.2829370145910843, -295.4964954922735387 ) ) ;
#62029=CARTESIAN_POINT ( 'NONE',  ( 36.35323700740005393, -289.5285428368790690, -279.3010128509669130 ) ) ;
#62030=CARTESIAN_POINT ( 'NONE',  ( -43.00533730372855956, -281.6046660885201618, -343.8870566229210795 ) ) ;
#62031=CARTESIAN_POINT ( 'NONE',  ( -110.4585283288373603, -279.9710658600658917, -262.4444270426106982 ) ) ;
#62032=CARTESIAN_POINT ( 'NONE',  ( -68.05759070136770106, -277.9590193362187165, -336.6660712836229550 ) ) ;
#62033=CARTESIAN_POINT ( 'NONE',  ( -106.1635557968894830, -288.9115243562584965, -304.1204208501723087 ) ) ;
#62034=CARTESIAN_POINT ( 'NONE',  ( -114.0464436410450304, -285.2878630260869386, -275.7167332093262075 ) ) ;
#62035=CARTESIAN_POINT ( 'NONE',  ( -7.372890411164062741, -286.9269605338669180, -199.4426914957515180 ) ) ;
#62036=CARTESIAN_POINT ( 'NONE',  ( -3.619494781854760479, -282.7608040994583689, -335.1193343622798011 ) ) ;
#62039=CARTESIAN_POINT ( 'NONE',  ( -112.9566010682902260, -292.4731156138514052, -265.5974813395214369 ) ) ;
#62040=CARTESIAN_POINT ( 'NONE',  ( 15.11232305184130986, -291.4583789379362884, -214.5938944494969576 ) ) ;
#62041=CARTESIAN_POINT ( 'NONE',  ( -35.37202290742290245, -273.1361887275465961, -197.1397696029900146 ) ) ;
#62042=CARTESIAN_POINT ( 'NONE',  ( -98.19888279386984209, -295.2724616619329936, -317.3687355040290186 ) ) ;
#62044=CARTESIAN_POINT ( 'NONE',  ( -27.99944512366560190, -290.6526229892918423, -197.2111179662545055 ) ) ;
#62045=CARTESIAN_POINT ( 'NONE',  ( -0.2695385665357618032, -292.7921766650520112, -334.4791762848074086 ) ) ;
#62046=CARTESIAN_POINT ( 'NONE',  ( -96.07689904917971546, -291.1424740988965709, -314.3969356862227755 ) ) ;
#62048=CARTESIAN_POINT ( 'NONE',  ( -86.06528975434426343, -291.7272892425266377, -327.4469619221611651 ) ) ;
#62049=CARTESIAN_POINT ( 'NONE',  ( 35.64796997533456846, -291.3218501120428527, -252.4018170869155711 ) ) ;
#62050=CARTESIAN_POINT ( 'NONE',  ( -42.29319392709419390, -297.1147268780757713, -345.2101703396592143 ) ) ;
#62051=CARTESIAN_POINT ( 'NONE',  ( 15.18995221619665159, -287.7579702751744435, -219.3333417226234019 ) ) ;
#62052=CARTESIAN_POINT ( 'NONE',  ( 35.68489131738341769, -277.2943622563719259, -251.7728488861518770 ) ) ;
#62053=CARTESIAN_POINT ( 'NONE',  ( -54.05961776822132947, -276.0569862513044654, -345.1718827872111319 ) ) ;
#62054=CARTESIAN_POINT ( 'NONE',  ( -57.33782044864310024, -296.9977701891475022, -196.1148932415864010 ) ) ;
#62055=CARTESIAN_POINT ( 'NONE',  ( 27.64593417192388358, -274.2701701604668756, -305.8882705148748187 ) ) ;
#62056=CARTESIAN_POINT ( 'NONE',  ( -102.0517628199790607, -277.1262178491890040, -233.5654391325326458 ) ) ;
#62057=CARTESIAN_POINT ( 'NONE',  ( -83.45188516503738185, -274.6085259240046526, -213.2561152291569897 ) ) ;
#62058=CARTESIAN_POINT ( 'NONE',  ( -96.44692722915402783, -276.2997146413598557, -318.4753461207172904 ) ) ;
#62060=CARTESIAN_POINT ( 'NONE',  ( -109.6848670926615199, -273.3465166235943684, -259.5097327623465731 ) ) ;
#62062=CARTESIAN_POINT ( 'NONE',  ( -7.592971423522123509, -286.6842587832781533, -339.6095800180198125 ) ) ;
#62063=CARTESIAN_POINT ( 'NONE',  ( -0.5444365648930986623, -274.3891671933071734, -207.2992319510063339 ) ) ;
#62064=CARTESIAN_POINT ( 'NONE',  ( 10.22794607770020825, -288.4168270954785953, -330.9775148117028039 ) ) ;
#62065=CARTESIAN_POINT ( 'NONE',  ( -28.98369397163828509, -288.6158184824765272, -346.9384032508500013 ) ) ;
#62066=CARTESIAN_POINT ( 'NONE',  ( -110.9921122315878961, -298.3283609184059628, -286.2992359406437686 ) ) ;
#62067=CARTESIAN_POINT ( 'NONE',  ( 13.58431560165681873, -292.3372727882368167, -325.2643101730104149 ) ) ;
#62068=CARTESIAN_POINT ( 'NONE',  ( 33.02916626481745510, -280.3549935369239847, -239.5050005480852917 ) ) ;
#62070=CARTESIAN_POINT ( 'NONE',  ( 0.7186967764620975085, -278.5594444973312420, -205.7211978478155743 ) ) ;
#62072=CARTESIAN_POINT ( 'NONE',  ( -80.65412912895703812, -288.4489736295436160, -329.6794475771482098 ) ) ;
#62076=CARTESIAN_POINT ( 'NONE',  ( -94.05253960020942827, -289.2327514533021713, -221.2807620594313107 ) ) ;
#62077=CARTESIAN_POINT ( 'NONE',  ( -68.59406182953972575, -275.1539859244670083, -203.6090115705580388 ) ) ;
#62078=CARTESIAN_POINT ( 'NONE',  ( 8.867009346162118888, -283.8574427595171983, -331.2163680439941231 ) ) ;
#62079=CARTESIAN_POINT ( 'NONE',  ( -30.64117882779282453, -296.1557469306057442, -195.0081571552323680 ) ) ;
#62080=CARTESIAN_POINT ( 'NONE',  ( -99.03103644794438765, -284.0116487594899013, -309.4868380060408981 ) ) ;
#62081=CARTESIAN_POINT ( 'NONE',  ( -79.20506578675527010, -274.9005666449506293, -209.7778623687303536 ) ) ;
#62082=CARTESIAN_POINT ( 'NONE',  ( -21.90991519230977502, -275.0578397395916568, -198.8456529409580185 ) ) ;
#62084=CARTESIAN_POINT ( 'NONE',  ( 16.41112582024762645, -284.2891632781772842, -322.7386447316769136 ) ) ;
#62085=CARTESIAN_POINT ( 'NONE',  ( -104.6581200486104564, -271.8624684733359231, -241.2027911472995072 ) ) ;
#62088=CARTESIAN_POINT ( 'NONE',  ( 36.36906994952523320, -293.6669782561295960, -292.8065455158306349 ) ) ;
#62089=CARTESIAN_POINT ( 'NONE',  ( -71.96299850839584167, -287.5719105631092702, -204.2308487871470675 ) ) ;
#62091=CARTESIAN_POINT ( 'NONE',  ( -37.37352853689063181, -280.5523547857346784, -350.3611179825600175 ) ) ;
#62092=CARTESIAN_POINT ( 'NONE',  ( -70.24117767164770498, -276.6718362368798694, -339.8145869037289799 ) ) ;
#62093=CARTESIAN_POINT ( 'NONE',  ( -93.02230521703508259, -288.2345469052291378, -322.4574771044648855 ) ) ;
#62094=CARTESIAN_POINT ( 'NONE',  ( -6.950020853574732982, -284.1660580654667001, -337.5095568509012764 ) ) ;
#62096=CARTESIAN_POINT ( 'NONE',  ( -81.40494210337182324, -279.4209719899201332, -329.8287959066548751 ) ) ;
#62097=CARTESIAN_POINT ( 'NONE',  ( -35.89203359648348624, -284.4596045891721019, -346.7711549717291746 ) ) ;
#62098=CARTESIAN_POINT ( 'NONE',  ( -109.1115541506471089, -283.1446389177461356, -285.7902715749403910 ) ) ;
#62099=CARTESIAN_POINT ( 'NONE',  ( 22.08545324069955029, -282.9252805419743595, -224.5864126013558462 ) ) ;
#62100=CARTESIAN_POINT ( 'NONE',  ( 34.72100672315269065, -275.3756129215487363, -243.2324194187547732 ) ) ;
#62101=CARTESIAN_POINT ( 'NONE',  ( -97.93022228132296902, -277.7502395641690214, -317.8798615246766417 ) ) ;
#62103=CARTESIAN_POINT ( 'NONE',  ( -17.81977085263746119, -296.7185993498702601, -342.1957090408149611 ) ) ;
#62104=CARTESIAN_POINT ( 'NONE',  ( 120.8395553409046528, -299.5541904835127980, -198.3007743052732792 ) ) ;
#62107=CARTESIAN_POINT ( 'NONE',  ( -95.57745119697061398, -294.0290686025301170, -318.8467793659812628 ) ) ;
#62108=CARTESIAN_POINT ( 'NONE',  ( 26.69348107032817552, -274.5784373497921820, -235.0777681290601606 ) ) ;
#62109=CARTESIAN_POINT ( 'NONE',  ( -57.32248995891848864, -298.8799711926172336, -196.2637697770827288 ) ) ;
#62111=CARTESIAN_POINT ( 'NONE',  ( 5.291014087692663459, -288.3975249725554022, -209.7969619150125880 ) ) ;
#62112=CARTESIAN_POINT ( 'NONE',  ( -99.43294874909099690, -297.4783453547395879, -314.8052961785273851 ) ) ;
#62113=CARTESIAN_POINT ( 'NONE',  ( -68.05282981142289600, -296.6515943598110994, -340.5382882952985142 ) ) ;
#62114=CARTESIAN_POINT ( 'NONE',  ( -106.8055689469605056, -292.1872567177941278, -298.3352901802377346 ) ) ;
#62115=CARTESIAN_POINT ( 'NONE',  ( -21.78912545874645090, -278.2516332011640543, -197.1085981219497683 ) ) ;
#62116=CARTESIAN_POINT ( 'NONE',  ( -84.36596313540567849, -281.3198302490087599, -212.5879455084361496 ) ) ;
#62117=CARTESIAN_POINT ( 'NONE',  ( -110.7876024639096215, -294.4751420900199150, -282.4860356768754741 ) ) ;
#62118=CARTESIAN_POINT ( 'NONE',  ( -31.70417339903574572, -284.8421506815395787, -345.9289464635023705 ) ) ;
#62119=CARTESIAN_POINT ( 'NONE',  ( 32.97033250405802107, -286.1985792965833184, -249.5696582420201821 ) ) ;
#62120=CARTESIAN_POINT ( 'NONE',  ( 203.7290947897051581, 292.0717063975089332, -83.07512796522757981 ) ) ;
#62122=CARTESIAN_POINT ( 'NONE',  ( -19.80666994010270443, -285.9505902719658934, -199.4766330582423279 ) ) ;
#62124=CARTESIAN_POINT ( 'NONE',  ( 37.56658326136570736, -282.8390015065806438, -286.8608395150154706 ) ) ;
#62125=CARTESIAN_POINT ( 'NONE',  ( -67.06999895155297509, -273.9846896992810343, -203.6517256073753970 ) ) ;
#62126=CARTESIAN_POINT ( 'NONE',  ( -29.48830978224716759, -284.9444597675504838, -194.1618202281204049 ) ) ;
#62127=CARTESIAN_POINT ( 'NONE',  ( 20.87979170948735330, -281.8158129399775476, -220.3103626705945146 ) ) ;
#62129=CARTESIAN_POINT ( 'NONE',  ( -69.68626442336800153, -281.1541948377401923, -201.2343622537274541 ) ) ;
#62130=CARTESIAN_POINT ( 'NONE',  ( 24.57220920650583551, -281.2773509347484264, -224.6182264856387292 ) ) ;
#62131=CARTESIAN_POINT ( 'NONE',  ( -21.39648532958014826, -280.3380690714490129, -340.3683826091709079 ) ) ;
#62132=CARTESIAN_POINT ( 'NONE',  ( 204.3871895515903248, 295.4036489450776344, -54.00000000003383605 ) ) ;
#62134=CARTESIAN_POINT ( 'NONE',  ( -88.60735235691279854, -275.3316383907295517, -215.7753651459944422 ) ) ;
#62135=CARTESIAN_POINT ( 'NONE',  ( 173.3098281514585040, 243.5254134702760211, -179.4893097426693771 ) ) ;
#62136=CARTESIAN_POINT ( 'NONE',  ( 30.47740036453139822, -279.1594020060218782, -239.0535628851937702 ) ) ;
#62137=CARTESIAN_POINT ( 'NONE',  ( 38.64185183667098755, -295.2754350200712565, -267.4527298032458589 ) ) ;
#62138=CARTESIAN_POINT ( 'NONE',  ( -93.16559935020049465, -295.2307301742486061, -317.5778107881095593 ) ) ;
#62139=CARTESIAN_POINT ( 'NONE',  ( -40.62351505635263038, -291.5196022840518708, -193.4795093570113806 ) ) ;
#62142=CARTESIAN_POINT ( 'NONE',  ( -111.0286456077016908, -294.8716545358064991, -290.5809191632632178 ) ) ;
#62143=CARTESIAN_POINT ( 'NONE',  ( 27.07551686922100842, -285.4635472034391910, -234.2445319275487918 ) ) ;
#62144=CARTESIAN_POINT ( 'NONE',  ( 11.72985059892390503, -294.6020353073982392, -214.5893274861555255 ) ) ;
#62146=CARTESIAN_POINT ( 'NONE',  ( -106.6331183573653618, -285.5417501068845922, -295.0062926344954235 ) ) ;
#62148=CARTESIAN_POINT ( 'NONE',  ( 37.55700646905299322, -294.7051800203935272, -287.2432111417434726 ) ) ;
#62149=CARTESIAN_POINT ( 'NONE',  ( -45.64023667855260413, -283.6523760868956288, -343.0008779458037225 ) ) ;
#62150=CARTESIAN_POINT ( 'NONE',  ( -113.2612344036847816, -295.2138434393336297, -280.9596399593287401 ) ) ;
#62151=CARTESIAN_POINT ( 'NONE',  ( -95.54530537253452849, -292.0339637288088284, -220.1762832888179560 ) ) ;
#62152=CARTESIAN_POINT ( 'NONE',  ( -109.4183958288736278, -291.3868878979236001, -243.2931504269986647 ) ) ;
#62153=CARTESIAN_POINT ( 'NONE',  ( -94.94925562757360638, -290.0868885829125929, -315.2184576338083275 ) ) ;
#62154=ORIENTED_EDGE ( 'NONE', *, *, #37168, .F. ) ;
#62156=CARTESIAN_POINT ( 'NONE',  ( -76.42442664383926854, -297.4289509700955705, -335.3285831218125850 ) ) ;
#62157=CARTESIAN_POINT ( 'NONE',  ( 7.645358440375352949, -297.2891121358272244, -193.8640699574521022 ) ) ;
#62158=CARTESIAN_POINT ( 'NONE',  ( -43.75980346380193708, -279.0279412631193736, -197.3571999250343083 ) ) ;
#62160=CARTESIAN_POINT ( 'NONE',  ( 37.88654482869483076, -274.8571148510014837, -254.1669164176647655 ) ) ;
#62161=CARTESIAN_POINT ( 'NONE',  ( -80.11489271843522886, -295.9410960898944722, -210.3514375431061580 ) ) ;
#62162=CARTESIAN_POINT ( 'NONE',  ( -10.79049564206102474, -278.5626062800440650, -339.6857097285516147 ) ) ;
#62163=CARTESIAN_POINT ( 'NONE',  ( -16.26770224259139397, -272.4669118267210592, -199.1263901020467699 ) ) ;
#62164=CARTESIAN_POINT ( 'NONE',  ( 4.052911788363070755, -295.6855722450789585, -330.9714851510532299 ) ) ;
#62165=CARTESIAN_POINT ( 'NONE',  ( -58.00501875971919219, -298.8585124888522842, -200.0244039849526985 ) ) ;
#62167=CARTESIAN_POINT ( 'NONE',  ( -103.8941601764363156, -297.6648574020217666, -307.5797208467027986 ) ) ;
#62168=CARTESIAN_POINT ( 'NONE',  ( -20.98205275373969059, -296.2563299801637413, -195.2000046196192216 ) ) ;
#62169=CARTESIAN_POINT ( 'NONE',  ( -37.55856933149814836, -292.7008172564774213, -197.2470453172807936 ) ) ;
#62170=CARTESIAN_POINT ( 'NONE',  ( -110.5573194955301233, -289.2237879378496928, -262.9551746229625451 ) ) ;
#62172=CARTESIAN_POINT ( 'NONE',  ( 39.31971637931158625, -276.1261469021078483, -276.8844700492973629 ) ) ;
#62173=CARTESIAN_POINT ( 'NONE',  ( -64.57075795394921158, -273.8532170690698990, -202.6159731627336953 ) ) ;
#62174=CARTESIAN_POINT ( 'NONE',  ( -40.95529554936418037, -281.9868107631513112, -195.0796935737309639 ) ) ;
#62175=CARTESIAN_POINT ( 'NONE',  ( -78.90594608002184884, -282.2847860487191269, -334.5928214507551957 ) ) ;
#62176=CARTESIAN_POINT ( 'NONE',  ( -67.67604294049554881, -276.7884704012433872, -341.0232749900562226 ) ) ;
#62177=CARTESIAN_POINT ( 'NONE',  ( -106.6820819435996981, -284.0604918745594887, -246.8677466567403656 ) ) ;
#62178=CARTESIAN_POINT ( 'NONE',  ( 23.60547888971174046, -280.1498402576630724, -314.3769318207641277 ) ) ;
#62179=CARTESIAN_POINT ( 'NONE',  ( -59.63702038127579641, -272.3325145182950564, -200.1772273572711356 ) ) ;
#62180=CARTESIAN_POINT ( 'NONE',  ( -83.89852987808885132, -279.6912897503808040, -329.2267780005162194 ) ) ;
#62183=CARTESIAN_POINT ( 'NONE',  ( -37.58166642864219398, -296.2890518265519972, -194.3748268903636358 ) ) ;
#62185=CARTESIAN_POINT ( 'NONE',  ( -111.9020112372838298, -280.6794707972761671, -260.4358155944297550 ) ) ;
#62188=CARTESIAN_POINT ( 'NONE',  ( -68.56859125762616713, -285.3794172014340234, -339.1807501379173004 ) ) ;
#62191=CARTESIAN_POINT ( 'NONE',  ( -0.9852217125672030340, -286.5697797886974172, -336.0174713571342977 ) ) ;
#62193=CARTESIAN_POINT ( 'NONE',  ( -34.30001684065561562, -293.8079815565538411, -343.6951392033938077 ) ) ;
#62194=CARTESIAN_POINT ( 'NONE',  ( -75.36864611930531055, -287.7044805633208853, -334.1319720925894217 ) ) ;
#62195=CARTESIAN_POINT ( 'NONE',  ( 138.4517698930976621, 181.0451598467585939, -241.7086681466011271 ) ) ;
#62196=CARTESIAN_POINT ( 'NONE',  ( -108.7819560547770976, -294.2553407669294643, -293.3612140365323171 ) ) ;
#62197=CARTESIAN_POINT ( 'NONE',  ( -26.69848670156409298, -284.6649274932117919, -194.7473310146409915 ) ) ;
#62198=CARTESIAN_POINT ( 'NONE',  ( 26.25870376865906408, -283.6620765842991432, -307.8978119973273806 ) ) ;
#62199=CARTESIAN_POINT ( 'NONE',  ( 14.48677208943751360, -279.0087569188588077, -214.7213415024717449 ) ) ;
#62200=CARTESIAN_POINT ( 'NONE',  ( -71.17275951027551173, -289.5117698735611498, -335.0626382165620498 ) ) ;
#62201=CARTESIAN_POINT ( 'NONE',  ( -30.22331026722054048, -281.5691033478844361, -197.0662206807416794 ) ) ;
#62202=CARTESIAN_POINT ( 'NONE',  ( -71.02509121847224094, -280.3986100589895045, -205.4006291246342641 ) ) ;
#62203=CARTESIAN_POINT ( 'NONE',  ( 24.98251055041723490, -288.9610914447134746, -227.9812658396922984 ) ) ;
#62205=CARTESIAN_POINT ( 'NONE',  ( -109.1666012014669604, -272.9053404859841407, -242.4621692476984549 ) ) ;
#62206=CARTESIAN_POINT ( 'NONE',  ( -107.2599707565800173, -292.8747889406675426, -244.0746472647838061 ) ) ;
#62208=CARTESIAN_POINT ( 'NONE',  ( 36.57525178469696669, -289.6233781216987495, -234.7283546768995564 ) ) ;
#62210=CARTESIAN_POINT ( 'NONE',  ( -3.572137588767112071, -274.6074148396185706, -337.5293354932284160 ) ) ;
#62212=CARTESIAN_POINT ( 'NONE',  ( -93.11793476103430578, -294.2367479262866823, -322.2980845871433644 ) ) ;
#62213=CARTESIAN_POINT ( 'NONE',  ( -98.49564652132110609, -296.6144729756389324, -230.2922925035794890 ) ) ;
#62214=CARTESIAN_POINT ( 'NONE',  ( 16.53092511624394589, -289.7893199401704010, -320.7194814161749719 ) ) ;
#62215=CARTESIAN_POINT ( 'NONE',  ( -33.42042955250219194, -284.7622921157316682, -344.2832530809398008 ) ) ;
#62217=CARTESIAN_POINT ( 'NONE',  ( -44.85729453125748734, -293.3841869319554689, -194.2683338550819769 ) ) ;
#62218=CARTESIAN_POINT ( 'NONE',  ( -77.86092985218138551, -290.8991469505770056, -335.3189054361162675 ) ) ;
#62219=CARTESIAN_POINT ( 'NONE',  ( -8.753996469251035251, -288.4263100696713309, -201.0093461868228530 ) ) ;
#62220=CARTESIAN_POINT ( 'NONE',  ( -86.80634661059910684, -279.5529981287041323, -211.2810381927050685 ) ) ;
#62221=CARTESIAN_POINT ( 'NONE',  ( -97.92297538639601839, -295.2443516461229365, -225.1817723909588267 ) ) ;
#62222=CARTESIAN_POINT ( 'NONE',  ( -88.32312638259294602, -283.5763024639051650, -328.1375482307881271 ) ) ;
#62223=CARTESIAN_POINT ( 'NONE',  ( 30.20020228012788976, -277.0026696384394427, -239.4317089190700756 ) ) ;
#62224=CARTESIAN_POINT ( 'NONE',  ( 17.36665895637874613, -283.4090924074130839, -226.6919474004047572 ) ) ;
#62225=CARTESIAN_POINT ( 'NONE',  ( -37.15419900124892649, -275.1893838209671799, -346.1385384650019432 ) ) ;
#62227=CARTESIAN_POINT ( 'NONE',  ( 29.36808933716896064, -281.4621798982450400, -300.2811593355019681 ) ) ;
#62228=CARTESIAN_POINT ( 'NONE',  ( -98.47720799253986002, -279.1390823461998707, -316.5395301165770547 ) ) ;
#62229=CARTESIAN_POINT ( 'NONE',  ( -87.58685523860694389, -284.4297309891798591, -212.2541756122675167 ) ) ;
#62230=CARTESIAN_POINT ( 'NONE',  ( 34.28325986600994923, -295.0694365392945997, -251.7106723720840478 ) ) ;
#62231=CARTESIAN_POINT ( 'NONE',  ( 36.50484994859345989, -276.9146598850203986, -251.5694320710709633 ) ) ;
#62232=CARTESIAN_POINT ( 'NONE',  ( 36.80313869455389408, -276.6297516045722773, -251.4973656980204453 ) ) ;
#62234=CARTESIAN_POINT ( 'NONE',  ( 26.76573876936310725, -275.8633748726827548, -305.3843496052797946 ) ) ;
#62235=CARTESIAN_POINT ( 'NONE',  ( -76.59865566483408372, -297.5784857718181797, -334.1311727324882099 ) ) ;
#62236=CARTESIAN_POINT ( 'NONE',  ( -111.2272806913039034, -282.7058103662303097, -258.4079084322780773 ) ) ;
#62237=CARTESIAN_POINT ( 'NONE',  ( 37.74162592964486862, -293.0058193798369075, -253.3244163209103590 ) ) ;
#62238=CARTESIAN_POINT ( 'NONE',  ( 37.76484639844176883, -288.9887539159295216, -257.4218512884738743 ) ) ;
#62239=CARTESIAN_POINT ( 'NONE',  ( 25.11841529032293963, -291.9445315659485800, -231.8855585433479973 ) ) ;
#62241=CARTESIAN_POINT ( 'NONE',  ( -7.404202894446433980, -291.0118138316977934, -200.0450368370763385 ) ) ;
#62242=CARTESIAN_POINT ( 'NONE',  ( -38.89377451390601692, -291.6988662010831490, -197.3564705143335800 ) ) ;
#62244=CARTESIAN_POINT ( 'NONE',  ( -96.14515598847482636, -290.9663796717601372, -319.6120225732753397 ) ) ;
#62245=CARTESIAN_POINT ( 'NONE',  ( -68.53617384229421816, -279.9638232903423614, -204.3384529608535161 ) ) ;
#62246=CARTESIAN_POINT ( 'NONE',  ( -73.12411131233280059, -296.5098503811270234, -202.4710213324340202 ) ) ;
#62247=CARTESIAN_POINT ( 'NONE',  ( -26.64350433382007211, -286.8361129305421855, -194.1574349464007980 ) ) ;
#62248=CARTESIAN_POINT ( 'NONE',  ( -33.73256646877940312, -286.4296850851458771, -193.4669150424163320 ) ) ;
#62249=CARTESIAN_POINT ( 'NONE',  ( 9.925612838762564394, -282.7134201884878735, -326.0862959525955489 ) ) ;
#62250=CARTESIAN_POINT ( 'NONE',  ( -107.9691066305277900, -262.3882541908849930, -317.6205384922552071 ) ) ;
#62251=CARTESIAN_POINT ( 'NONE',  ( -64.72634346049389364, -182.0697847625480676, -361.3728755866533220 ) ) ;
#62252=CARTESIAN_POINT ( 'NONE',  ( 178.4789072661037324, 251.8278643662533227, -164.2970973383132218 ) ) ;
#62254=CARTESIAN_POINT ( 'NONE',  ( 30.42374033854767390, -275.1195021424367155, -298.0720726600726493 ) ) ;
#62255=CARTESIAN_POINT ( 'NONE',  ( -6.157571474655167520, -275.5527995923927165, -336.7208263011962117 ) ) ;
#62256=CARTESIAN_POINT ( 'NONE',  ( -113.7129358895308258, -296.1765255516202160, -261.0358163016437629 ) ) ;
#62257=CARTESIAN_POINT ( 'NONE',  ( -87.60137065885514573, -230.3911852031648095, -345.0379683109082976 ) ) ;
#62259=CARTESIAN_POINT ( 'NONE',  ( 33.26494053643585147, -273.8583473668449528, -240.7623666379177507 ) ) ;
#62260=CARTESIAN_POINT ( 'NONE',  ( -107.2710463876148168, -274.6303226597171943, -246.1152823722235610 ) ) ;
#62262=CARTESIAN_POINT ( 'NONE',  ( -71.27843577842449463, -274.6942235811085311, -201.5876457377155475 ) ) ;
#62264=CARTESIAN_POINT ( 'NONE',  ( 32.72720757791289259, -287.7703440749824040, -249.6207029913926760 ) ) ;
#62265=CARTESIAN_POINT ( 'NONE',  ( -101.4878145052344962, -296.7964816164920308, -312.7590373905729848 ) ) ;
#62266=CARTESIAN_POINT ( 'NONE',  ( -111.9074532997213964, -296.8064591108852710, -289.3741227362523887 ) ) ;
#62267=CARTESIAN_POINT ( 'NONE',  ( 8.229822628023377717, -294.5755523371689151, -327.4544666561328086 ) ) ;
#62269=CARTESIAN_POINT ( 'NONE',  ( 20.64162240762772882, -278.1366667372432744, -318.8095287819680266 ) ) ;
#62271=CARTESIAN_POINT ( 'NONE',  ( 37.61896585007993110, -280.8422093359563974, -252.9704270377555702 ) ) ;
#62272=CARTESIAN_POINT ( 'NONE',  ( 17.61972441668371658, -277.1824857078469222, -318.7809730813240208 ) ) ;
#62273=CARTESIAN_POINT ( 'NONE',  ( -48.32506735422127520, -278.9500972431155219, -345.6029948150822975 ) ) ;
#62274=CARTESIAN_POINT ( 'NONE',  ( -88.12270743237529302, -275.7788769931800061, -326.0360324193958377 ) ) ;
#62275=CARTESIAN_POINT ( 'NONE',  ( -92.96470659711444284, -273.7179062915847680, -222.9701921779713416 ) ) ;
#62276=CARTESIAN_POINT ( 'NONE',  ( -63.79764198944837261, -293.9785674031145959, -339.0843076935979070 ) ) ;
#62278=CARTESIAN_POINT ( 'NONE',  ( 15.11478982441561669, -281.2608826231216312, -214.0046946443562774 ) ) ;
#62279=CARTESIAN_POINT ( 'NONE',  ( -104.4429021786955190, -279.1050151316099459, -241.6134452446196121 ) ) ;
#62280=CARTESIAN_POINT ( 'NONE',  ( -31.87882060011769525, -287.6695438861580669, -346.7249042943355448 ) ) ;
#62281=CARTESIAN_POINT ( 'NONE',  ( -96.25820521449435319, -275.1895370121113729, -223.9515706693634058 ) ) ;
#62283=CARTESIAN_POINT ( 'NONE',  ( -61.31755919635303798, -288.5688196649106203, -339.4824599019588618 ) ) ;
#62284=CARTESIAN_POINT ( 'NONE',  ( -99.25722516425169317, -284.5084307304362028, -224.6689048950553911 ) ) ;
#62285=CARTESIAN_POINT ( 'NONE',  ( 19.25495086030587188, -280.4604971436399978, -318.0755753502187986 ) ) ;
#62286=CARTESIAN_POINT ( 'NONE',  ( 34.80478897936795590, -280.3174573717301996, -284.9247679092526937 ) ) ;
#62287=CARTESIAN_POINT ( 'NONE',  ( -111.5329183808475761, -282.5533272256720352, -276.4420167760204663 ) ) ;
#62288=CARTESIAN_POINT ( 'NONE',  ( 37.64345686072064723, -289.5118462650171978, -267.2091669108579595 ) ) ;
#62289=CARTESIAN_POINT ( 'NONE',  ( -110.7892205932846110, -279.7533807707761753, -270.6548755915363245 ) ) ;
#62290=CARTESIAN_POINT ( 'NONE',  ( -114.0438498160389287, -273.6021560138187851, -270.3744733279939965 ) ) ;
#62291=CARTESIAN_POINT ( 'NONE',  ( -55.72390417005674124, -293.8158264148777334, -197.5951775443839438 ) ) ;
#62292=CARTESIAN_POINT ( 'NONE',  ( -72.39344909896090030, -275.7493423561646750, -337.7948328303848484 ) ) ;
#62293=CARTESIAN_POINT ( 'NONE',  ( 32.19770090373580018, -276.5022262521604262, -292.9036194482267206 ) ) ;
#62294=CARTESIAN_POINT ( 'NONE',  ( -2.461704542035739962, -284.5919402306911365, -336.9450074551469925 ) ) ;
#62296=CARTESIAN_POINT ( 'NONE',  ( -59.57969948219484024, -291.2581091499336026, -342.5745902756821124 ) ) ;
#62297=CARTESIAN_POINT ( 'NONE',  ( -43.72117530519366824, -293.1325884930290613, -345.1021094493497117 ) ) ;
#62298=CARTESIAN_POINT ( 'NONE',  ( -29.46929581545144217, -285.3466380642558988, -193.9269366848511140 ) ) ;
#62299=CARTESIAN_POINT ( 'NONE',  ( -93.14823700134739681, -289.6327189066530536, -222.0695984494056745 ) ) ;
#62301=CARTESIAN_POINT ( 'NONE',  ( 35.19111776844810180, -274.3961652592252562, -282.5102284564745787 ) ) ;
#62302=CARTESIAN_POINT ( 'NONE',  ( -66.56076885441905233, -293.5785622425982524, -338.6041506293255452 ) ) ;
#62305=CARTESIAN_POINT ( 'NONE',  ( -113.6965737442166358, -289.0214237832831827, -271.2016239971042069 ) ) ;
#62306=CARTESIAN_POINT ( 'NONE',  ( -111.1908020677759765, -286.1447916747094951, -270.9356432036289561 ) ) ;
#62307=CARTESIAN_POINT ( 'NONE',  ( 4.974180390718086819, -286.7285756609774694, -333.4748270157836600 ) ) ;
#62308=CARTESIAN_POINT ( 'NONE',  ( -109.5542299297093933, -285.7920277897581514, -284.5288792083869680 ) ) ;
#62310=CARTESIAN_POINT ( 'NONE',  ( -10.70067695605413149, -287.2115324048096454, -202.2090452305314727 ) ) ;
#62311=CARTESIAN_POINT ( 'NONE',  ( 10.06405564870831704, -294.6812964441883764, -211.7184013412460502 ) ) ;
#62312=CARTESIAN_POINT ( 'NONE',  ( -112.9444886269548505, -276.6167081423948275, -271.5606673702270086 ) ) ;
#62314=CARTESIAN_POINT ( 'NONE',  ( 12.69409406138459673, -276.7094762035383724, -328.8603794417296058 ) ) ;
#62316=CARTESIAN_POINT ( 'NONE',  ( 32.01253885703746960, -291.2425904643599210, -240.3727247253076769 ) ) ;
#62317=CARTESIAN_POINT ( 'NONE',  ( -53.76047810733812327, -279.8471846651020201, -195.0774075345661913 ) ) ;
#62318=CARTESIAN_POINT ( 'NONE',  ( -83.35431795387779630, -297.6657019384484784, -329.2035771400176145 ) ) ;
#62320=DIRECTION ( 'NONE',  ( -1.000000000000000000, -0.000000000000000000, -0.000000000000000000 ) ) ;
#62321=CARTESIAN_POINT ( 'NONE',  ( -60.11565295431227440, -284.4354952349557379, -200.4855818491412549 ) ) ;
#62322=CARTESIAN_POINT ( 'NONE',  ( -111.5857481016875994, -276.7243928445810184, -267.8431239756961872 ) ) ;
#62323=CARTESIAN_POINT ( 'NONE',  ( 35.73472859122758649, -279.3346401917989397, -253.4275152831069704 ) ) ;
#62325=CARTESIAN_POINT ( 'NONE',  ( 37.81265487832424554, -273.8643681791504036, -257.0753435488216496 ) ) ;
#62326=CARTESIAN_POINT ( 'NONE',  ( -105.3656794337780980, -277.5432412610031747, -297.1310807648108607 ) ) ;
#62327=CIRCLE ( 'NONE', #53249, 5.654241149514405151 ) ;
#62328=CARTESIAN_POINT ( 'NONE',  ( 35.59117400344509008, -294.9342921106934341, -259.8015903632006030 ) ) ;
#62329=CARTESIAN_POINT ( 'NONE',  ( -33.91527017283922874, -279.0146453053664004, -193.7468106495906568 ) ) ;
#62330=CARTESIAN_POINT ( 'NONE',  ( -45.10379467290600530, -296.0939746842353202, -343.2345443711770372 ) ) ;
#62331=CARTESIAN_POINT ( 'NONE',  ( -101.1477144667957759, -298.4264383768374387, -228.1224375188270983 ) ) ;
#62332=CARTESIAN_POINT ( 'NONE',  ( -88.12421900725803425, -297.1507672713754005, -217.8488087742622383 ) ) ;
#62333=CARTESIAN_POINT ( 'NONE',  ( -50.05206480986360873, -293.8902599599312566, -196.3932482834451605 ) ) ;
#62334=CARTESIAN_POINT ( 'NONE',  ( -65.87933393469943155, -285.8556564122085888, -198.8305073732281585 ) ) ;
#62335=CARTESIAN_POINT ( 'NONE',  ( 38.08996893649335647, -273.5947266555241981, -262.7287153336583287 ) ) ;
#62336=CARTESIAN_POINT ( 'NONE',  ( 24.14092809487967628, -288.0027541231248165, -316.7172009849429060 ) ) ;
#62337=CARTESIAN_POINT ( 'NONE',  ( -49.43261822015174545, -281.8771459112280695, -196.7020621924338002 ) ) ;
#62338=CARTESIAN_POINT ( 'NONE',  ( 17.99546967229176175, -287.2930537704831409, -318.4079180155812310 ) ) ;
#62339=CARTESIAN_POINT ( 'NONE',  ( -110.9112672685687642, -288.3639759336571160, -285.0043701770196094 ) ) ;
#62340=CARTESIAN_POINT ( 'NONE',  ( 197.9738562182569694, 291.4636489450775798, -54.00000000000003553 ) ) ;
#62341=CARTESIAN_POINT ( 'NONE',  ( 5.875982438000423969, -287.9562129263955512, -329.3327402905377994 ) ) ;
#62343=CARTESIAN_POINT ( 'NONE',  ( 24.07408639797774441, -283.1082028506222059, -316.4145801655532750 ) ) ;
#62344=CARTESIAN_POINT ( 'NONE',  ( -69.51358087324699397, -290.6977654384454013, -200.6489710628453338 ) ) ;
#62345=CARTESIAN_POINT ( 'NONE',  ( 38.73191045385964770, -283.2183039940754838, -275.5855336575278898 ) ) ;
#62346=CARTESIAN_POINT ( 'NONE',  ( -45.23923029067531587, -281.2694123057322031, -194.2103242226465625 ) ) ;
#62347=CARTESIAN_POINT ( 'NONE',  ( 13.92316989062081056, -282.1419199862598362, -322.4025980071550634 ) ) ;
#62348=CARTESIAN_POINT ( 'NONE',  ( 21.40665245858204102, -276.9115181653517652, -223.7183545380449061 ) ) ;
#62349=CARTESIAN_POINT ( 'NONE',  ( -94.65157633605407739, -295.8542301174773002, -321.8062239351966127 ) ) ;
#62350=CARTESIAN_POINT ( 'NONE',  ( -91.80985505795345603, -287.8533485217014913, -321.4764849362650807 ) ) ;
#62351=CARTESIAN_POINT ( 'NONE',  ( -91.40468242996172421, -272.0558860269956085, -220.7005550978051076 ) ) ;
#62354=CARTESIAN_POINT ( 'NONE',  ( -96.24110771372400563, -285.8435248029016975, -315.9030550999602269 ) ) ;
#62355=CARTESIAN_POINT ( 'NONE',  ( -50.40130165100462278, -296.2946767704760873, -345.9856021812352083 ) ) ;
#62356=CARTESIAN_POINT ( 'NONE',  ( -4.774309824762142718, -283.2628284514468078, -335.8077203189584452 ) ) ;
#62358=CARTESIAN_POINT ( 'NONE',  ( 21.54240632842849124, -275.2757235098295610, -319.6103029564845883 ) ) ;
#62359=CARTESIAN_POINT ( 'NONE',  ( -97.38917831966689675, -291.8478637371387663, -222.3234957470463655 ) ) ;
#62360=CARTESIAN_POINT ( 'NONE',  ( -112.9769329981831305, -282.6250433140344853, -275.6082475782509391 ) ) ;
#62361=CARTESIAN_POINT ( 'NONE',  ( 33.30330949930436191, -293.4956629715330791, -239.7829083196810416 ) ) ;
#62362=CARTESIAN_POINT ( 'NONE',  ( -97.36386924569266910, -290.3059262529394005, -311.9694601597855694 ) ) ;
#62365=CARTESIAN_POINT ( 'NONE',  ( -101.7143074437604326, -254.4836201735207624, -324.1852191778334031 ) ) ;
#62366=CARTESIAN_POINT ( 'NONE',  ( -92.91321726759508692, -285.3518244813142815, -322.6728513055225562 ) ) ;
#62367=CARTESIAN_POINT ( 'NONE',  ( -20.25526795762938548, -280.3380690714491266, -345.3683826091709648 ) ) ;
#62369=CARTESIAN_POINT ( 'NONE',  ( 18.72190567208880196, -281.1408569231107322, -317.6151018503476848 ) ) ;
#62370=CARTESIAN_POINT ( 'NONE',  ( -20.13496104240586249, -276.5037457805761960, -345.4469640604518190 ) ) ;
#62371=CARTESIAN_POINT ( 'NONE',  ( -101.0413650427625925, -281.0817090332643602, -230.9890489329771981 ) ) ;
#62372=CARTESIAN_POINT ( 'NONE',  ( 169.5298778015222467, 230.0351857080673597, -191.1287857711722893 ) ) ;
#62373=CARTESIAN_POINT ( 'NONE',  ( 1.093412870664322689, -279.1290506314940671, -204.2603646273037157 ) ) ;
#62374=CARTESIAN_POINT ( 'NONE',  ( -111.9642018374680390, -282.5293493250019310, -273.6868261862858844 ) ) ;
#62375=CARTESIAN_POINT ( 'NONE',  ( -35.52496992298293321, -299.8347340750885905, -194.3739090059161754 ) ) ;
#62376=CARTESIAN_POINT ( 'NONE',  ( 34.96774734480509039, -293.9066831759812999, -259.9049117941014515 ) ) ;
#62377=ORIENTED_EDGE ( 'NONE', *, *, #26867, .T. ) ;
#62378=CARTESIAN_POINT ( 'NONE',  ( -102.8415333438375825, -289.6879897458907180, -236.9166185282000470 ) ) ;
#62379=CARTESIAN_POINT ( 'NONE',  ( -62.36497023060947242, -278.0205783917635927, -343.1301319342535976 ) ) ;
#62380=CARTESIAN_POINT ( 'NONE',  ( 35.02050904442798895, -275.4251344293097077, -260.7324792587318143 ) ) ;
#62381=CARTESIAN_POINT ( 'NONE',  ( 37.87649728430607610, -274.6602989537010444, -285.3182329698734065 ) ) ;
#62383=CARTESIAN_POINT ( 'NONE',  ( -112.1851880641518591, -270.6236085282212684, -264.7831444951723938 ) ) ;
#62388=B_SPLINE_CURVE_WITH_KNOTS ( 'NONE', 3,
 ( #65758, #80379, #29747, #1779, #52433, #9330, #73304, #868, #8867, #30663, #59565, #88415, #87469, #22616, #38212, #60031, #23565, #67126, #51491, #8415, #37294, #66200, #16454, #59088 ),
 .UNSPECIFIED., .F., .F.,
 ( 4, 2, 2, 2, 2, 2, 2, 2, 2, 2, 2, 4 ),
 ( 0.000000000000000000, 0.06250000000000000000, 0.1250000000000000000, 0.2500000000000000000, 0.3750000000000000000, 0.5000000000000000000, 0.6250000000000000000, 0.7500000000000000000, 0.8125000000000000000, 0.8750000000000000000, 0.9375000000000000000, 1.000000000000000000 ),
 .UNSPECIFIED. ) ;
#62390=CARTESIAN_POINT ( 'NONE',  ( 14.15155330994995708, -283.3880706110204528, -322.6118245859823332 ) ) ;
#62391=CARTESIAN_POINT ( 'NONE',  ( 31.48419404549470002, -283.7315166635507353, -302.6871839486440194 ) ) ;
#62392=CARTESIAN_POINT ( 'NONE',  ( -110.3294487919163487, -283.9654290596298551, -265.4501027286298722 ) ) ;
#62393=CARTESIAN_POINT ( 'NONE',  ( -54.15578548279486171, -275.6713989405343455, -342.2729103553705841 ) ) ;
#62394=CARTESIAN_POINT ( 'NONE',  ( 34.95808848542053227, -283.1941045221067839, -253.5205107959050963 ) ) ;
#62395=CARTESIAN_POINT ( 'NONE',  ( -29.66022299610497015, -275.4331448678845504, -343.7044069217980109 ) ) ;
#62398=CARTESIAN_POINT ( 'NONE',  ( 19.22865231693831589, -275.9737913726957004, -223.7347166756766228 ) ) ;
#62401=CARTESIAN_POINT ( 'NONE',  ( -62.00549743442884676, -280.5424472260224888, -197.5323689875521325 ) ) ;
#62404=CARTESIAN_POINT ( 'NONE',  ( -49.17555213449553264, -287.7634478231784669, -195.4733212497631314 ) ) ;
#62405=CARTESIAN_POINT ( 'NONE',  ( -69.80489281814210756, -294.6881784786021399, -335.9259168298979716 ) ) ;
#62406=CARTESIAN_POINT ( 'NONE',  ( -99.79234140298613909, -289.3049936502433752, -315.2527150401634231 ) ) ;
#62407=CARTESIAN_POINT ( 'NONE',  ( 34.70178695010155678, -285.5706038365906920, -253.3442598677782485 ) ) ;
#62408=CARTESIAN_POINT ( 'NONE',  ( 36.24421497864828012, -286.1360139554283819, -271.0596974885449981 ) ) ;
#62409=CARTESIAN_POINT ( 'NONE',  ( -94.20416234706810599, -289.4552210628647799, -222.9637676311234316 ) ) ;
#62410=CARTESIAN_POINT ( 'NONE',  ( -99.35836934679360866, -285.2165302608587467, -309.7126131320366085 ) ) ;
#62411=CARTESIAN_POINT ( 'NONE',  ( -37.15812013368570632, -275.0496619246393948, -345.3736166798979639 ) ) ;
#62412=CARTESIAN_POINT ( 'NONE',  ( -21.13405276700971669, -284.6566193647917089, -195.9047375949826062 ) ) ;
#62413=CARTESIAN_POINT ( 'NONE',  ( -62.20663637494677545, -299.7289374520364049, -199.6028280573134737 ) ) ;
#62414=CARTESIAN_POINT ( 'NONE',  ( 17.04307828501119104, -284.8245188364803084, -218.3984126723973134 ) ) ;
#62415=CARTESIAN_POINT ( 'NONE',  ( -49.19174876028269239, -280.8386729497715351, -198.0908973176059646 ) ) ;
#62416=CARTESIAN_POINT ( 'NONE',  ( -10.20096042202992237, -290.6988631622684238, -340.4568288000978669 ) ) ;
#62419=CARTESIAN_POINT ( 'NONE',  ( -67.62615583989033041, -297.3665570891805032, -339.5865897590450686 ) ) ;
#62421=CARTESIAN_POINT ( 'NONE',  ( -108.3297018451442426, -276.8668976356065627, -246.0004692778863102 ) ) ;
#62422=CARTESIAN_POINT ( 'NONE',  ( 23.85284377214213336, -292.1285575222582906, -223.8702619586156857 ) ) ;
#62423=CARTESIAN_POINT ( 'NONE',  ( -109.2520098646687359, -295.1685481382422722, -253.7675116425085946 ) ) ;
#62424=CARTESIAN_POINT ( 'NONE',  ( 29.42767931392143410, -279.8240132139270600, -239.5292703110461048 ) ) ;
#62425=CARTESIAN_POINT ( 'NONE',  ( 8.231418428188186809, -272.7610376279750426, -211.5019210804418321 ) ) ;
#62426=CARTESIAN_POINT ( 'NONE',  ( 29.94826031768689134, -295.2622187699211054, -299.9128472022380834 ) ) ;
#62427=CARTESIAN_POINT ( 'NONE',  ( 31.95455697924148097, -289.6233781216988064, -236.9535640164627353 ) ) ;
#62428=CARTESIAN_POINT ( 'NONE',  ( -99.45551301604132277, -294.4385924375687864, -314.7737509732767762 ) ) ;
#62429=CARTESIAN_POINT ( 'NONE',  ( -16.80261486949788718, -293.0304192470185853, -343.5738033895680132 ) ) ;
#62430=CARTESIAN_POINT ( 'NONE',  ( -98.80157278307707713, -292.5353156550247036, -229.7955823903595274 ) ) ;
#62432=CARTESIAN_POINT ( 'NONE',  ( -90.88431813285613714, -292.0704497226151375, -220.4848967948219354 ) ) ;
#62434=CARTESIAN_POINT ( 'NONE',  ( -44.29314567706702377, -281.1596327508506192, -345.4472234807956852 ) ) ;
#62435=CARTESIAN_POINT ( 'NONE',  ( -6.041630355387678009, -292.4753562337936614, -204.3980705274468335 ) ) ;
#62436=CARTESIAN_POINT ( 'NONE',  ( -3.657608455576050410, -280.4844072356609104, -201.1051240153441029 ) ) ;
#62437=CARTESIAN_POINT ( 'NONE',  ( -94.38633936651712020, -283.5163525430716049, -322.0687089692151517 ) ) ;
#62438=CARTESIAN_POINT ( 'NONE',  ( -5.023155395706768722, -286.6255172733480094, -337.8558592423685241 ) ) ;
#62439=CARTESIAN_POINT ( 'NONE',  ( -59.33632811234290472, -281.4793595096010108, -341.3172225293729980 ) ) ;
#62440=CARTESIAN_POINT ( 'NONE',  ( 3.467677775316871269, -279.0697180669168915, -205.8215476114294518 ) ) ;
#62441=CARTESIAN_POINT ( 'NONE',  ( 25.30059580559607824, -285.8844116762513181, -226.0955590603487053 ) ) ;
#62443=CARTESIAN_POINT ( 'NONE',  ( 34.85440377562154879, -295.3527501364723094, -285.7241969558337473 ) ) ;
#62444=CARTESIAN_POINT ( 'NONE',  ( -53.98508847651596909, -278.6869110234774780, -344.9914994142048954 ) ) ;
#62445=CARTESIAN_POINT ( 'NONE',  ( -96.11254663185624736, -277.6114152121239158, -313.7188419019598200 ) ) ;
#62446=CARTESIAN_POINT ( 'NONE',  ( -95.66230492618028336, -291.3979140027301469, -220.0646567606551969 ) ) ;
#62448=CARTESIAN_POINT ( 'NONE',  ( 8.318817480842051637, -280.5125548425954776, -330.5643681182293108 ) ) ;
#62449=CARTESIAN_POINT ( 'NONE',  ( 31.05239761278816246, -292.2623130835193592, -244.1760871081505684 ) ) ;
#62451=CARTESIAN_POINT ( 'NONE',  ( -104.1870360930141430, -294.1010451502096998, -304.4859149042151785 ) ) ;
#62455=CARTESIAN_POINT ( 'NONE',  ( 35.26734991781270168, -293.1726653885826863, -278.9239710856059560 ) ) ;
#62456=CARTESIAN_POINT ( 'NONE',  ( 133.0872704186301405, -299.5541904835127980, -195.3611179825600175 ) ) ;
#62457=CARTESIAN_POINT ( 'NONE',  ( -109.1418805571601069, -288.0523547857347353, -270.3284710469131937 ) ) ;
#62458=CARTESIAN_POINT ( 'NONE',  ( -94.95860783121142390, -272.4391540804525675, -219.5236242650188103 ) ) ;
#62459=CARTESIAN_POINT ( 'NONE',  ( 7.829418448290626387, -278.8009198773373782, -209.4692856207271063 ) ) ;
#62460=VECTOR ( 'NONE', #59286, 999.9999999999998863 ) ;
#62461=CARTESIAN_POINT ( 'NONE',  ( -32.35539466067025671, -287.4289301519967239, -194.0038480387398749 ) ) ;
#62462=CARTESIAN_POINT ( 'NONE',  ( 24.23720895448933632, -287.9275498323750071, -309.5661936832856895 ) ) ;
#62464=CARTESIAN_POINT ( 'NONE',  ( -111.0452528469028124, -280.1043867483486451, -267.9042783526909943 ) ) ;
#62465=CARTESIAN_POINT ( 'NONE',  ( -102.9241848702152282, -294.0964316652198249, -306.0091823762008403 ) ) ;
#62466=CARTESIAN_POINT ( 'NONE',  ( -97.21513662511344478, -297.7114223709497765, -313.8930348137300257 ) ) ;
#62467=CARTESIAN_POINT ( 'NONE',  ( -95.59749364166030716, -276.7223577774606724, -315.0085482345307355 ) ) ;
#62469=CARTESIAN_POINT ( 'NONE',  ( 53.56078642086819031, -298.8278332737911001, -193.3871885607800323 ) ) ;
#62470=CARTESIAN_POINT ( 'NONE',  ( -59.08687513482454534, -291.2557567528447748, -341.6080858073236186 ) ) ;
#62471=CARTESIAN_POINT ( 'NONE',  ( 18.81219702445331166, -294.4441009831222118, -218.8520872178545744 ) ) ;
#62472=CARTESIAN_POINT ( 'NONE',  ( 201.9720043525299218, 292.2277401595099491, -53.99999999997594102 ) ) ;
#62474=CARTESIAN_POINT ( 'NONE',  ( -23.75810946330653906, -289.5255355364519687, -342.2417055962533823 ) ) ;
#62477=CARTESIAN_POINT ( 'NONE',  ( -112.5037681141233037, -297.0000969593267541, -286.6084661711859667 ) ) ;
#62478=CARTESIAN_POINT ( 'NONE',  ( -112.7746364397447110, -288.7886372312765957, -262.7373097285047834 ) ) ;
#62479=CARTESIAN_POINT ( 'NONE',  ( -31.91564562775961633, -298.4516268701335093, -193.3819643928579524 ) ) ;
#62483=CARTESIAN_POINT ( 'NONE',  ( -8.477295177102565304, -290.2012511749268810, -341.0120317553232212 ) ) ;
#62484=CARTESIAN_POINT ( 'NONE',  ( -117.3417001280813707, -275.0519495502701943, -270.3929463913696054 ) ) ;
#62485=CARTESIAN_POINT ( 'NONE',  ( 23.31738787103862975, -281.5332207163203293, -317.6453586990783720 ) ) ;
#62486=CARTESIAN_POINT ( 'NONE',  ( -78.06764539347322795, -287.5039227357324876, -207.5188477820374260 ) ) ;
#62487=CARTESIAN_POINT ( 'NONE',  ( -33.73682970312665219, -284.6714157335118216, -194.0354263511844977 ) ) ;
#62488=CARTESIAN_POINT ( 'NONE',  ( -62.62575788680646838, -271.7221775669246995, -199.9285626617074172 ) ) ;
#62489=CARTESIAN_POINT ( 'NONE',  ( -31.24569009509668049, -276.0498759169886966, -196.1582407838954794 ) ) ;
#62490=CARTESIAN_POINT ( 'NONE',  ( -93.51414036032699073, -287.9483848098208796, -319.2845846413326854 ) ) ;
#62491=CARTESIAN_POINT ( 'NONE',  ( -96.08147876313722691, -279.7596982539052419, -318.2347852238114001 ) ) ;
#62494=CARTESIAN_POINT ( 'NONE',  ( -3.149092476846345523, -280.5170641353806786, -205.8499202825576049 ) ) ;
#62495=CARTESIAN_POINT ( 'NONE',  ( 35.66730939899011332, -280.9492747752598234, -274.0458426340898654 ) ) ;
#62496=CARTESIAN_POINT ( 'NONE',  ( -37.11402287224021990, -278.1289949830828618, -347.0646758699858765 ) ) ;
#62497=CARTESIAN_POINT ( 'NONE',  ( 38.88137406026387310, -280.4492902885523904, -278.4917145783999217 ) ) ;
#62498=CARTESIAN_POINT ( 'NONE',  ( 119.9181164563876649, 148.9434379163483015, -261.0995976656233779 ) ) ;
#62499=CARTESIAN_POINT ( 'NONE',  ( 38.49328721732177883, -276.3429173315491312, -258.3653461316740731 ) ) ;
#62501=CARTESIAN_POINT ( 'NONE',  ( -110.3792060108426796, -274.3542079634458446, -248.0844052571740690 ) ) ;
#62502=CARTESIAN_POINT ( 'NONE',  ( -54.42813229853333468, -291.7662352645558599, -345.3683826091709648 ) ) ;
#62505=CARTESIAN_POINT ( 'NONE',  ( 30.77749032570432064, -288.9944198009672505, -297.5905662195247601 ) ) ;
#62506=CARTESIAN_POINT ( 'NONE',  ( 34.12714280562018843, -289.6443356662788347, -296.3247671150632527 ) ) ;
#62507=CARTESIAN_POINT ( 'NONE',  ( -110.2249809973208841, -289.8181481158409838, -276.6304047091149414 ) ) ;
#62508=CARTESIAN_POINT ( 'NONE',  ( -73.57848248213724673, -285.0924594981007658, -202.4314823492213691 ) ) ;
#62509=CARTESIAN_POINT ( 'NONE',  ( 26.54924896572594406, -23.55631650609774752, -345.1007383875407299 ) ) ;
#62510=CARTESIAN_POINT ( 'NONE',  ( 35.35864716923569517, -279.7863996783452762, -257.6686036887648470 ) ) ;
#62511=CARTESIAN_POINT ( 'NONE',  ( 35.19803604602822134, -289.2079317681412363, -254.5860693470918363 ) ) ;
#62512=CARTESIAN_POINT ( 'NONE',  ( 12.37027135513538312, -280.8245057082112908, -324.7617396909143963 ) ) ;
#62513=CARTESIAN_POINT ( 'NONE',  ( -83.76210701367267575, -280.7149475510340721, -213.3181424732781863 ) ) ;
#62514=CARTESIAN_POINT ( 'NONE',  ( -3.833662056930598361, -277.0898906721354820, -335.2856882657222855 ) ) ;
#62515=CARTESIAN_POINT ( 'NONE',  ( -96.09642893474666892, -288.6820020519545551, -319.5331786034835204 ) ) ;
#62516=CARTESIAN_POINT ( 'NONE',  ( -114.1793417686187126, -285.3595991801640821, -269.9928149620623685 ) ) ;
#62517=CARTESIAN_POINT ( 'NONE',  ( -105.7265730229388652, -284.5884055529612624, -305.7340591338137301 ) ) ;
#62518=CARTESIAN_POINT ( 'NONE',  ( 35.14004538967056845, -281.8388114359333372, -279.4561300441198455 ) ) ;
#62521=CARTESIAN_POINT ( 'NONE',  ( -99.03918675619182466, -293.0044606163714320, -226.3869707419946451 ) ) ;
#62523=CARTESIAN_POINT ( 'NONE',  ( -33.54696690536734849, -290.7838132249228806, -193.9484340011192103 ) ) ;
#62524=CARTESIAN_POINT ( 'NONE',  ( 35.61374299019288969, -274.5194967565503248, -263.4102978018960926 ) ) ;
#62525=CARTESIAN_POINT ( 'NONE',  ( -114.1325566424810916, -295.8385838841359146, -275.3245156865346530 ) ) ;
#62526=CARTESIAN_POINT ( 'NONE',  ( -72.94509993043601526, -290.0515824854518314, -205.7816483703690835 ) ) ;
#62527=CARTESIAN_POINT ( 'NONE',  ( 2.091012644759666639, -292.7566170396970620, -333.0559432045100152 ) ) ;
#62529=CARTESIAN_POINT ( 'NONE',  ( -31.82628276922260824, -290.1862258789201974, -343.6015698292261504 ) ) ;
#62532=CARTESIAN_POINT ( 'NONE',  ( -79.39749743985044006, -291.6197162172724688, -332.5230426707244078 ) ) ;
#62533=CARTESIAN_POINT ( 'NONE',  ( -25.28968528822433726, -290.2052931969116116, -196.1669311322207534 ) ) ;
#62534=CARTESIAN_POINT ( 'NONE',  ( 36.67595890380260215, -295.7086654504139460, -282.5382331042629858 ) ) ;
#62535=CARTESIAN_POINT ( 'NONE',  ( 19.69089987937389807, -287.8457026778626187, -224.3989954509325457 ) ) ;
#62536=CARTESIAN_POINT ( 'NONE',  ( 36.80222480147381248, -295.7116295172220362, -282.7967236884273916 ) ) ;
#62537=AXIS2_PLACEMENT_3D ( 'NONE', #3349, #16175, #37469 ) ;
#62538=CARTESIAN_POINT ( 'NONE',  ( -2.093673719876190553, -276.4963916838688078, -203.7579390827001191 ) ) ;
#62539=CARTESIAN_POINT ( 'NONE',  ( 12.43490360822420016, -275.1713669133288249, -328.5873872945156222 ) ) ;
#62540=CARTESIAN_POINT ( 'NONE',  ( -31.91341839994286289, -297.3156647644431132, -193.5233109628402417 ) ) ;
#62541=CARTESIAN_POINT ( 'NONE',  ( 10.29943968133824406, -274.6240121980960112, -327.0029382979065531 ) ) ;
#62542=CARTESIAN_POINT ( 'NONE',  ( -6.144032942095575045, -278.5451416597068715, -202.7600743682178290 ) ) ;
#62543=CARTESIAN_POINT ( 'NONE',  ( -33.79891809001208713, -299.4125882376109189, -196.8671507568475931 ) ) ;
#62545=CARTESIAN_POINT ( 'NONE',  ( -63.76373908956360737, -296.8286521384384855, -339.0973470259114606 ) ) ;
#62547=CARTESIAN_POINT ( 'NONE',  ( -100.0404418221979768, -297.8737701061027678, -232.5601944838269048 ) ) ;
#62549=CARTESIAN_POINT ( 'NONE',  ( 24.48738717028066958, -286.1550089500391891, -313.5270067797571869 ) ) ;
#62550=CARTESIAN_POINT ( 'NONE',  ( -105.4154717941531203, -272.7393905257599158, -243.8595651865568925 ) ) ;
#62552=CARTESIAN_POINT ( 'NONE',  ( 28.69854607509536848, -287.0346374543865977, -230.6642725504785574 ) ) ;
#62553=CARTESIAN_POINT ( 'NONE',  ( -107.7137651166459733, -289.8191206141484599, -301.6934681854449423 ) ) ;
#62554=CARTESIAN_POINT ( 'NONE',  ( -110.0420831950332854, -298.7880005354153354, -250.3422926058365192 ) ) ;
#62555=CARTESIAN_POINT ( 'NONE',  ( 35.55568063452456329, -291.7702765593687104, -287.3290290903524919 ) ) ;
#62556=CARTESIAN_POINT ( 'NONE',  ( 37.82883484982344413, -280.5489738526259771, -254.3748957718820520 ) ) ;
#62558=CARTESIAN_POINT ( 'NONE',  ( -48.49081814431468018, -277.9101904052724876, -196.1428057292681615 ) ) ;
#62561=CARTESIAN_POINT ( 'NONE',  ( -23.72648930226850794, -287.6693453420479045, -342.5362998687483014 ) ) ;
#62563=CARTESIAN_POINT ( 'NONE',  ( -67.14663747770097757, -287.4425783543860007, -339.2400677067841457 ) ) ;
#62564=CARTESIAN_POINT ( 'NONE',  ( -84.60261042645456087, -298.9889732991502456, -213.6124007350129546 ) ) ;
#62565=CARTESIAN_POINT ( 'NONE',  ( 37.57148526252345277, -283.1671408037443030, -285.4150526582834573 ) ) ;
#62566=CARTESIAN_POINT ( 'NONE',  ( -112.4289050837386412, -270.7395577891506377, -261.9215771874306711 ) ) ;
#62567=CARTESIAN_POINT ( 'NONE',  ( -105.2139348631828568, -284.1909844448757099, -297.3754695694228189 ) ) ;
#62568=CARTESIAN_POINT ( 'NONE',  ( 0.9033207881293309205, -275.9986143485042476, -207.4906695028003583 ) ) ;
#62570=CARTESIAN_POINT ( 'NONE',  ( 37.53427269006324707, -283.6182716941420381, -275.4978649170241169 ) ) ;
#62571=CARTESIAN_POINT ( 'NONE',  ( -68.40108027298184368, -272.5546139077140424, -203.9429883882090166 ) ) ;
#62574=CARTESIAN_POINT ( 'NONE',  ( 35.45330800551266748, -293.0672954734139353, -245.1021611932829956 ) ) ;
#62575=CARTESIAN_POINT ( 'NONE',  ( -111.7329616175136096, -286.4527453021829047, -276.5082323215308406 ) ) ;
#62576=DIRECTION ( 'NONE',  ( 1.000000000000000000, 0.000000000000000000, 0.000000000000000000 ) ) ;
#62577=CARTESIAN_POINT ( 'NONE',  ( -111.2869819898779866, -275.6237833571633473, -305.9350535429201159 ) ) ;
#62578=CARTESIAN_POINT ( 'NONE',  ( -82.45974247071691821, -276.8482542599046496, -332.5585542255541895 ) ) ;
#62579=CARTESIAN_POINT ( 'NONE',  ( -67.75351038329525011, -287.8445335521758466, -340.2292953879033348 ) ) ;
#62580=CARTESIAN_POINT ( 'NONE',  ( -104.7396718578417278, -285.6749583615194297, -300.1641573799864773 ) ) ;
#62581=CARTESIAN_POINT ( 'NONE',  ( -24.12695981134176648, -278.6413819671305987, -343.2373515770221957 ) ) ;
#62582=CARTESIAN_POINT ( 'NONE',  ( -110.9191536318844555, -285.7171071123252091, -290.9757882353332548 ) ) ;
#62583=CARTESIAN_POINT ( 'NONE',  ( -91.97079509739259606, -282.6491644875575275, -319.3983216736398276 ) ) ;
#62584=CARTESIAN_POINT ( 'NONE',  ( -60.37133141458019026, -281.7538362498117408, -198.9296222287348428 ) ) ;
#62585=CARTESIAN_POINT ( 'NONE',  ( -52.54769881529375652, -274.0293594243011057, -194.8230518923121508 ) ) ;
#62586=CARTESIAN_POINT ( 'NONE',  ( -14.59171986027598678, -276.5986751120722147, -343.9794226222867337 ) ) ;
#62587=CARTESIAN_POINT ( 'NONE',  ( -95.89119188554884943, -297.8365671294604340, -316.3314477254314170 ) ) ;
#62590=CARTESIAN_POINT ( 'NONE',  ( -112.3751245658655051, -294.8264108244034105, -259.7655397737052567 ) ) ;
#62591=CARTESIAN_POINT ( 'NONE',  ( 33.30009199879525283, -275.3058294070042962, -289.0085212044393757 ) ) ;
#62593=CARTESIAN_POINT ( 'NONE',  ( -113.1536202231119432, -273.8998112871589683, -259.0187801401784213 ) ) ;
#62594=CARTESIAN_POINT ( 'NONE',  ( -9.127565342238625590, -288.1863295667753846, -201.9227462911193243 ) ) ;
#62595=CARTESIAN_POINT ( 'NONE',  ( 38.53451918419519728, -294.9640340606317750, -261.7844428741461229 ) ) ;
#62596=CARTESIAN_POINT ( 'NONE',  ( 37.93219107720220507, -294.5786189762277445, -256.1537247561038839 ) ) ;
#62597=CARTESIAN_POINT ( 'NONE',  ( -87.16824830403565727, -293.3566860744488736, -214.4581739620171561 ) ) ;
#62598=APPLICATION_CONTEXT ( 'automotive_design' ) ;
#62599=CARTESIAN_POINT ( 'NONE',  ( -75.41719429619169546, -277.5434202745984749, -205.8788604737563332 ) ) ;
#62601=CARTESIAN_POINT ( 'NONE',  ( -111.0511528584513172, -280.6115305763220817, -259.5992293123894683 ) ) ;
#62602=CARTESIAN_POINT ( 'NONE',  ( -105.2603020961959288, -294.2280418209199979, -300.9565055639724847 ) ) ;
#62603=CARTESIAN_POINT ( 'NONE',  ( -69.91720982494362602, -285.3369331020471691, -338.7795976412631376 ) ) ;
#62604=CARTESIAN_POINT ( 'NONE',  ( -79.47575467268617899, -284.3887432512145210, -210.3075770829054534 ) ) ;
#62605=CARTESIAN_POINT ( 'NONE',  ( 187.0186979179691775, 261.8542818151678944, -152.7852267909635202 ) ) ;
#62607=CARTESIAN_POINT ( 'NONE',  ( -59.98115673316993224, -285.4172298914189696, -200.9381931568972846 ) ) ;
#62609=CARTESIAN_POINT ( 'NONE',  ( 38.36492379129992969, -282.7866394139171007, -282.6906722658144417 ) ) ;
#62611=CARTESIAN_POINT ( 'NONE',  ( -94.63194022947706685, -273.5241533536450333, -225.0851212955402332 ) ) ;
#62612=CARTESIAN_POINT ( 'NONE',  ( 19.99977743061145929, -285.6547891532740095, -219.4894533955281872 ) ) ;
#62614=CARTESIAN_POINT ( 'NONE',  ( -48.09770585449252422, -280.8598901677814865, -194.3000127185015060 ) ) ;
#62616=CARTESIAN_POINT ( 'NONE',  ( -42.40356559317686447, -281.5095189573240759, -194.2225254615520385 ) ) ;
#62617=CARTESIAN_POINT ( 'NONE',  ( -31.09032952305880215, -280.7804486691148895, -193.6649509313287751 ) ) ;
#62618=CARTESIAN_POINT ( 'NONE',  ( 34.45848030099739390, -279.0523547857346784, -270.3937649182068412 ) ) ;
#62619=CARTESIAN_POINT ( 'NONE',  ( -83.11721010220915673, -220.0893266087223878, -352.5837759202555048 ) ) ;
#62621=CARTESIAN_POINT ( 'NONE',  ( -49.19021291046425404, -275.9011149219318213, -196.4192727083408556 ) ) ;
#62622=CARTESIAN_POINT ( 'NONE',  ( -48.81378135290628251, -154.5565111508429936, -364.8478127054240190 ) ) ;
#62624=CARTESIAN_POINT ( 'NONE',  ( -7.315182385718625113, -278.4679806360489920, -202.0078707700635903 ) ) ;
#62625=CARTESIAN_POINT ( 'NONE',  ( 37.36517219576794702, -295.4891771257205164, -284.3188385113026015 ) ) ;
#62626=CARTESIAN_POINT ( 'NONE',  ( -80.22126148798015777, -294.9989459526885867, -329.5661505850004573 ) ) ;
#62627=CARTESIAN_POINT ( 'NONE',  ( -104.5531709379612977, -290.5456401981590489, -232.9158900536068586 ) ) ;
#62629=CARTESIAN_POINT ( 'NONE',  ( -95.14772181160688547, -294.4466649134712384, -320.3318109051483589 ) ) ;
#62630=CARTESIAN_POINT ( 'NONE',  ( 22.65371560706949694, -285.3568532875524397, -227.2983022257669461 ) ) ;
#62631=CARTESIAN_POINT ( 'NONE',  ( 11.11541274538510216, -296.2331216507247404, -326.5996607234354769 ) ) ;
#62632=CARTESIAN_POINT ( 'NONE',  ( -98.52684749151755739, -286.4286993546303961, -229.6472233002308769 ) ) ;
#62634=CARTESIAN_POINT ( 'NONE',  ( -19.45327542267640908, -293.2179284200299776, -195.6551127116425448 ) ) ;
#62635=CARTESIAN_POINT ( 'NONE',  ( 17.65531220614429486, -282.7301594279460915, -318.4580729391352634 ) ) ;
#62636=CARTESIAN_POINT ( 'NONE',  ( -79.27250989781455814, -294.3995770898573028, -334.4689639136826145 ) ) ;
#62638=CARTESIAN_POINT ( 'NONE',  ( -114.2075722186280871, -291.3799484244527775, -268.3691218432566075 ) ) ;
#62640=CARTESIAN_POINT ( 'NONE',  ( -72.15003753239496120, -292.0965833998297967, -201.7323437223217013 ) ) ;
#62641=CARTESIAN_POINT ( 'NONE',  ( 30.97384639226432057, -287.3737827200436072, -244.4893441569351182 ) ) ;
#62644=CARTESIAN_POINT ( 'NONE',  ( -68.99001483723060346, -297.3242864768307072, -339.2134581261443032 ) ) ;
#62645=CARTESIAN_POINT ( 'NONE',  ( -101.8912794902445569, -295.7787691208724254, -229.2922724131478276 ) ) ;
#62647=CARTESIAN_POINT ( 'NONE',  ( -54.53644206323097876, -278.8846278663562543, -199.1206287893511444 ) ) ;
#62648=VERTEX_POINT ( 'NONE', #19751 ) ;
#62649=CARTESIAN_POINT ( 'NONE',  ( 36.43266955204646962, -275.3345160659930002, -292.2449241545749601 ) ) ;
#62650=CARTESIAN_POINT ( 'NONE',  ( -73.16716868967206722, -296.0478441130085798, -205.9620220606466034 ) ) ;
#62651=CARTESIAN_POINT ( 'NONE',  ( -72.21381685430633013, -279.3789402764474517, -335.9101851615010901 ) ) ;
#62652=CARTESIAN_POINT ( 'NONE',  ( 32.28491054200005550, -273.3541066910371455, -244.6123206241607875 ) ) ;
#62653=CARTESIAN_POINT ( 'NONE',  ( -80.37524890574610481, -296.8551360638479082, -329.8190374161329146 ) ) ;
#62654=CARTESIAN_POINT ( 'NONE',  ( -92.98797878370415049, -298.3085114748986939, -222.6163635496660049 ) ) ;
#62655=DIRECTION ( 'NONE',  ( 0.000000000000000000, 0.000000000000000000, -1.000000000000000000 ) ) ;
#62656=CARTESIAN_POINT ( 'NONE',  ( -99.34554376769511919, -297.5583388518279548, -314.7440213026769129 ) ) ;
#62657=CARTESIAN_POINT ( 'NONE',  ( -9.919518414749692425, -296.3945003126609663, -195.2037656782123349 ) ) ;
#62658=CARTESIAN_POINT ( 'NONE',  ( -89.89535780959727163, -291.9367979451988617, -219.5476775119697095 ) ) ;
#62659=CARTESIAN_POINT ( 'NONE',  ( -96.25083141440101997, -288.5125514085958116, -314.4853188322464348 ) ) ;
#62661=CARTESIAN_POINT ( 'NONE',  ( 37.53343359844520677, -276.2666722501370486, -288.1165084887675221 ) ) ;
#62662=CARTESIAN_POINT ( 'NONE',  ( -79.74377151227155025, -297.7942008654942470, -210.9123852036024687 ) ) ;
#62663=CARTESIAN_POINT ( 'NONE',  ( -47.91351124033828768, -281.8983630975148458, -195.6984784909776067 ) ) ;
#62664=CARTESIAN_POINT ( 'NONE',  ( 30.29373307774961788, -279.7709726107038932, -234.4885631716222179 ) ) ;
#62666=CARTESIAN_POINT ( 'NONE',  ( -98.72707103111632421, -277.2828936139156895, -316.6984857735657215 ) ) ;
#62667=CARTESIAN_POINT ( 'NONE',  ( -42.95548625142242827, -282.3218397372677373, -343.3570973513015474 ) ) ;
#62668=CARTESIAN_POINT ( 'NONE',  ( 35.55955866712312741, -279.3172539801713583, -252.0462361592038576 ) ) ;
#62669=CARTESIAN_POINT ( 'NONE',  ( 21.16092167436010740, -273.5039061060537620, -225.6993780569914350 ) ) ;
#62670=CARTESIAN_POINT ( 'NONE',  ( -33.64081299148737259, -279.0057597512598022, -345.2824594583906332 ) ) ;
#62673=CARTESIAN_POINT ( 'NONE',  ( -36.53121673348384491, -296.3020323788277324, -194.3746836460879592 ) ) ;
#62675=CARTESIAN_POINT ( 'NONE',  ( 35.81363602509566135, -277.7742414619397664, -287.6887341515205776 ) ) ;
#62676=CARTESIAN_POINT ( 'NONE',  ( -77.61735700266031301, -271.5113161136116560, -207.0928628242538991 ) ) ;
#62678=CARTESIAN_POINT ( 'NONE',  ( -112.4694489270531790, -286.3694479938332620, -278.4317782485246653 ) ) ;
#62681=CARTESIAN_POINT ( 'NONE',  ( 36.93778946276158592, -285.6898161624158661, -281.0953053140264615 ) ) ;
#62684=CARTESIAN_POINT ( 'NONE',  ( -41.07468136076666809, -293.8950627699028928, -343.6758364479319425 ) ) ;
#62685=CARTESIAN_POINT ( 'NONE',  ( 27.45694720369125008, -285.2033015570177668, -234.0343339559310607 ) ) ;
#62687=CARTESIAN_POINT ( 'NONE',  ( 24.56995022601385870, -292.1264055027472750, -312.7833029782705694 ) ) ;
#62688=CARTESIAN_POINT ( 'NONE',  ( -35.14859000133749589, -284.5590708853400201, -194.0729462703540946 ) ) ;
#62689=CARTESIAN_POINT ( 'NONE',  ( -109.9225461035518236, -280.3266001598420303, -257.0021803742650945 ) ) ;
#62690=CARTESIAN_POINT ( 'NONE',  ( 31.06030618894929063, -288.3111701923981514, -235.8767120970426845 ) ) ;
#62691=CARTESIAN_POINT ( 'NONE',  ( 31.46516030874382253, -280.2118006691208052, -302.7276789914651545 ) ) ;
#62692=CARTESIAN_POINT ( 'NONE',  ( -73.54496383499513001, -289.5469024689942330, -333.7657786667729738 ) ) ;
#62696=CARTESIAN_POINT ( 'NONE',  ( -57.29023269278543751, -281.2149060249485615, -199.5272915704423156 ) ) ;
#62697=CARTESIAN_POINT ( 'NONE',  ( -54.54064568547437375, -280.6284318222396337, -199.1976369487024385 ) ) ;
#62698=CARTESIAN_POINT ( 'NONE',  ( 27.50150523380058587, -290.0430886122621246, -308.7507717873627939 ) ) ;
#62700=CARTESIAN_POINT ( 'NONE',  ( -13.06248678323646573, -274.3591155245477466, -197.2891000868189053 ) ) ;
#62701=CARTESIAN_POINT ( 'NONE',  ( -111.2479949310128262, -292.3957408418274326, -280.9266832379707921 ) ) ;
#62703=CARTESIAN_POINT ( 'NONE',  ( -111.2869819898779866, -299.4805209788416391, -234.7871824221999191 ) ) ;
#62705=CARTESIAN_POINT ( 'NONE',  ( -18.97273904071714057, -272.2877638656696035, -197.4197426308134595 ) ) ;
#62707=CARTESIAN_POINT ( 'NONE',  ( -83.71466702864759668, -294.0761168756562824, -330.8924283418914456 ) ) ;
#62708=CARTESIAN_POINT ( 'NONE',  ( -55.30272947268393580, -297.3225784875120894, -199.4893472628256461 ) ) ;
#62709=CARTESIAN_POINT ( 'NONE',  ( 34.38029981252815759, -289.2935358471168001, -287.2922277852051138 ) ) ;
#62711=CARTESIAN_POINT ( 'NONE',  ( 3.974218134601690711, -284.2478213355571484, -331.8313396177780987 ) ) ;
#62712=CARTESIAN_POINT ( 'NONE',  ( -93.14993036369341439, -291.2594594860639745, -322.6297629567361014 ) ) ;
#62713=CARTESIAN_POINT ( 'NONE',  ( -113.7579194640037059, -291.8204649465798184, -274.0839789721583770 ) ) ;
#62714=CARTESIAN_POINT ( 'NONE',  ( -80.47989825371161032, -287.4680793517698021, -208.9451122559017904 ) ) ;
#62715=CARTESIAN_POINT ( 'NONE',  ( -88.93301792798932581, -279.5172365102952767, -213.2005027640632306 ) ) ;
#62716=CARTESIAN_POINT ( 'NONE',  ( -110.5790831249054520, -294.3943480175670402, -289.0037384466583035 ) ) ;
#62717=CARTESIAN_POINT ( 'NONE',  ( -81.56329177113407525, -283.4686931348633152, -333.4612994687695391 ) ) ;
#62718=CARTESIAN_POINT ( 'NONE',  ( 23.49143409190629939, -277.9970424886916476, -312.9957969183646469 ) ) ;
#62719=CARTESIAN_POINT ( 'NONE',  ( -107.3417001280813565, -275.0519495502701943, -270.3929463913696054 ) ) ;
#62720=CARTESIAN_POINT ( 'NONE',  ( 19.10917282090019143, -274.4918965704873131, -321.2458266666068880 ) ) ;
#62721=DIRECTION ( 'NONE',  ( 0.000000000000000000, 0.000000000000000000, 1.000000000000000000 ) ) ;
#62722=CARTESIAN_POINT ( 'NONE',  ( 9.320655171656451188, -280.2209639846767004, -214.0758333842832144 ) ) ;
#62723=CARTESIAN_POINT ( 'NONE',  ( -77.59313309167708894, -278.7843671105878229, -335.5981379391097335 ) ) ;
#62724=CARTESIAN_POINT ( 'NONE',  ( -108.8050327343470087, -283.9689681205925922, -242.1842718366530676 ) ) ;
#62725=CARTESIAN_POINT ( 'NONE',  ( -68.24444091488061304, -293.4007669457184875, -203.0939779160814851 ) ) ;
#62726=CARTESIAN_POINT ( 'NONE',  ( 34.96430544092648773, -276.8444801812556761, -246.1474319583253418 ) ) ;
#62727=CARTESIAN_POINT ( 'NONE',  ( -63.40493579939095525, -275.0346729481839247, -198.4305541125026195 ) ) ;
#62728=DIRECTION ( 'NONE',  ( 0.000000000000000000, 0.000000000000000000, 1.000000000000000000 ) ) ;
#62729=CARTESIAN_POINT ( 'NONE',  ( 33.24165078580307409, -275.6314439061106896, -288.9888010991709280 ) ) ;
#62730=CARTESIAN_POINT ( 'NONE',  ( -72.97569013081923117, -297.5255909534118359, -336.1803567255897178 ) ) ;
#62731=CARTESIAN_POINT ( 'NONE',  ( -75.63696003311819993, -283.5396852724134646, -206.0688051045194413 ) ) ;
#62732=CARTESIAN_POINT ( 'NONE',  ( 36.26800391072323038, -292.9359667235247002, -247.8365588781600763 ) ) ;
#62733=CARTESIAN_POINT ( 'NONE',  ( 21.29930785552477346, -274.2096568668476380, -316.5669624958304667 ) ) ;
#62734=CARTESIAN_POINT ( 'NONE',  ( 36.93519571926441358, -288.9366319340879272, -253.2920122128685136 ) ) ;
#62735=CARTESIAN_POINT ( 'NONE',  ( 35.14149622896399450, -292.6209535354996092, -281.6641588051585927 ) ) ;
#62736=EDGE_LOOP ( 'NONE', ( #84262, #1766, #59810, #49462 ) ) ;
#62737=CARTESIAN_POINT ( 'NONE',  ( 22.65678290153533325, -291.4889667470666268, -223.0243669818048886 ) ) ;
#62738=CARTESIAN_POINT ( 'NONE',  ( -108.9603028792401602, -290.0301916667252726, -284.6680987808184682 ) ) ;
#62740=CARTESIAN_POINT ( 'NONE',  ( 16.07399888556184919, -287.8682476288912540, -215.3315295040999615 ) ) ;
#62741=CARTESIAN_POINT ( 'NONE',  ( -107.2485864805327509, -279.1646796863290092, -249.2633757501773175 ) ) ;
#62742=CARTESIAN_POINT ( 'NONE',  ( -97.17494649910651106, -294.8269232195877407, -318.3555977338385787 ) ) ;
#62743=CARTESIAN_POINT ( 'NONE',  ( -111.6249229510898573, -285.4551051145208476, -250.2783564824773066 ) ) ;
#62744=CARTESIAN_POINT ( 'NONE',  ( -110.6641110825146797, -284.5901271072877421, -293.8474538485443190 ) ) ;
#62745=CARTESIAN_POINT ( 'NONE',  ( 31.37593805074868314, -282.2160350820819872, -295.2082902698688827 ) ) ;
#62746=CARTESIAN_POINT ( 'NONE',  ( -31.25978362021906420, -124.2753969880052836, -364.3350065174659562 ) ) ;
#62747=CARTESIAN_POINT ( 'NONE',  ( -104.9959759434921978, -254.8895421021158825, -325.9787696571796687 ) ) ;
#62748=CARTESIAN_POINT ( 'NONE',  ( 195.4265002117133463, 282.6816008209588631, -110.3567886302177499 ) ) ;
#62749=CARTESIAN_POINT ( 'NONE',  ( 35.74888117987044467, -274.6937516812146214, -266.1398222809258414 ) ) ;
#62750=CARTESIAN_POINT ( 'NONE',  ( 33.88359738285667788, -274.7011203020184666, -287.7685829641801547 ) ) ;
#62751=CARTESIAN_POINT ( 'NONE',  ( -114.2763662760873586, -296.0693713248206222, -269.5968878146475731 ) ) ;
#62752=CARTESIAN_POINT ( 'NONE',  ( 202.3167528527534955, 289.8673209260633712, -82.47206762618345977 ) ) ;
#62753=CARTESIAN_POINT ( 'NONE',  ( 33.71994285826205129, -274.6005483994430847, -298.8506728662013643 ) ) ;
#62754=CARTESIAN_POINT ( 'NONE',  ( -106.3693248146888521, -274.6659015276296145, -243.5145553628732102 ) ) ;
#62756=CARTESIAN_POINT ( 'NONE',  ( -57.34001031339916210, -298.7415740595552052, -196.1919871017267951 ) ) ;
#62757=CARTESIAN_POINT ( 'NONE',  ( 32.37422570182891945, -288.3359240842070790, -292.3853954988765622 ) ) ;
#62758=CARTESIAN_POINT ( 'NONE',  ( -105.8091646611200360, -296.9035871611078505, -305.3547210544289214 ) ) ;
#62759=CARTESIAN_POINT ( 'NONE',  ( -97.30233451235987729, -297.6911090821166113, -222.1506499510646506 ) ) ;
#62760=CARTESIAN_POINT ( 'NONE',  ( -14.84841750065774768, -292.5185435159973508, -200.9129197256225723 ) ) ;
#62762=AXIS2_PLACEMENT_3D ( 'NONE', #51581, #16088, #8956 ) ;
#62763=CARTESIAN_POINT ( 'NONE',  ( 36.19617741455193993, -277.6942479999422062, -287.7805319183706843 ) ) ;
#62765=CARTESIAN_POINT ( 'NONE',  ( 39.35086845197975691, -280.9828769092899847, -264.2148322999018433 ) ) ;
#62767=CARTESIAN_POINT ( 'NONE',  ( -70.54881181584757144, -278.4425051179617867, -335.6351264557151808 ) ) ;
#62768=CARTESIAN_POINT ( 'NONE',  ( 5.321112988311692327, -278.2435700739887920, -333.2408316342586545 ) ) ;
#62769=CARTESIAN_POINT ( 'NONE',  ( -110.2427694978118922, -276.3277043791433130, -289.4864999557813690 ) ) ;
#62770=CARTESIAN_POINT ( 'NONE',  ( -108.8806052080202988, -297.4024165208856516, -255.2650157287278319 ) ) ;
#62771=CARTESIAN_POINT ( 'NONE',  ( -105.5145319565518349, -294.7586711984803287, -298.0710424915932322 ) ) ;
#62773=CARTESIAN_POINT ( 'NONE',  ( -35.34391528292362494, -280.5689106807918165, -193.4354714373812953 ) ) ;
#62774=CARTESIAN_POINT ( 'NONE',  ( -105.5150493298128254, -279.0691350487915088, -244.1159908687126290 ) ) ;
#62775=CARTESIAN_POINT ( 'NONE',  ( 22.88879431316950885, -286.8718589048248191, -317.5583218750372225 ) ) ;
#62776=CARTESIAN_POINT ( 'NONE',  ( -54.20913244213483750, -299.8361736911336948, -197.1114207096712221 ) ) ;
#62778=CARTESIAN_POINT ( 'NONE',  ( -58.74611564681632103, -288.5332085280372780, -340.3744068218875896 ) ) ;
#62779=CARTESIAN_POINT ( 'NONE',  ( -77.35104461874557558, -277.7477789645155895, -208.0326559401519830 ) ) ;
#62780=CARTESIAN_POINT ( 'NONE',  ( -95.24331146226769818, -277.7623556466783157, -224.9230235373411517 ) ) ;
#62781=CARTESIAN_POINT ( 'NONE',  ( -6.682297549938000181, -280.7263384966041713, -338.2080947406936957 ) ) ;
#62782=CARTESIAN_POINT ( 'NONE',  ( 31.47966560129664870, -289.1608091326579029, -240.4223764225739899 ) ) ;
#62783=CARTESIAN_POINT ( 'NONE',  ( -85.75755594294830075, -280.5689940042762487, -215.1974033733533531 ) ) ;
#62785=CARTESIAN_POINT ( 'NONE',  ( -85.25542858120036271, -293.3909305001070038, -212.5937928289431227 ) ) ;
#62786=CARTESIAN_POINT ( 'NONE',  ( -38.55160254141188148, -275.3069930335477693, -346.3381549943728714 ) ) ;
#62787=CARTESIAN_POINT ( 'NONE',  ( 18.39149936935317342, -276.8752284241597295, -317.6654850352001631 ) ) ;
#62788=CARTESIAN_POINT ( 'NONE',  ( 35.20864552864138375, -283.2995422316824943, -250.6533828290385486 ) ) ;
#62790=CARTESIAN_POINT ( 'NONE',  ( -101.0732837613175406, -291.9289619992819098, -311.0479882234540128 ) ) ;
#62791=CARTESIAN_POINT ( 'NONE',  ( -70.24715478444055350, -293.4855905774421103, -337.7711784007989877 ) ) ;
#62792=CARTESIAN_POINT ( 'NONE',  ( -112.2000957169564970, -283.9665355044935495, -253.0296601308724007 ) ) ;
#62794=CARTESIAN_POINT ( 'NONE',  ( -69.69305461488974629, -272.3018110807155949, -204.3714722606277121 ) ) ;
#62795=CARTESIAN_POINT ( 'NONE',  ( -17.07296494307979273, -290.4560539446659959, -198.8930388139336003 ) ) ;
#62797=CARTESIAN_POINT ( 'NONE',  ( -68.03198670781949886, -290.1363786050943645, -200.4840591525245941 ) ) ;
#62798=CARTESIAN_POINT ( 'NONE',  ( -54.96693575645529961, -287.4220216155817411, -198.6438069025912228 ) ) ;
#62799=CARTESIAN_POINT ( 'NONE',  ( 26.30144571015113897, -285.2393676315655284, -228.8457714103878402 ) ) ;
#62800=CARTESIAN_POINT ( 'NONE',  ( -70.26218259763309959, -287.0348579102766848, -204.5320406879389452 ) ) ;
#62802=CARTESIAN_POINT ( 'NONE',  ( -77.14547226032442495, -286.3067877318702017, -208.9148378088368645 ) ) ;
#62803=CARTESIAN_POINT ( 'NONE',  ( -7.857508652533764071, -294.4164281579045905, -200.9995072473832352 ) ) ;
#62804=CARTESIAN_POINT ( 'NONE',  ( 11.75014631036292911, -274.4564036757578833, -327.8006932644084941 ) ) ;
#62805=CARTESIAN_POINT ( 'NONE',  ( 38.47054325684204912, -275.7174719157262643, -256.9348643759292941 ) ) ;
#62806=CARTESIAN_POINT ( 'NONE',  ( 35.32614071337355455, -291.3669729121327236, -249.6088678844010929 ) ) ;
#62807=CARTESIAN_POINT ( 'NONE',  ( -113.2364877241909937, -278.7147260720351483, -257.3618404741212089 ) ) ;
#62808=CARTESIAN_POINT ( 'NONE',  ( -38.33954787723131830, -297.0446126150878285, -344.9992523805914857 ) ) ;
#62811=CARTESIAN_POINT ( 'NONE',  ( -70.18790354320688607, -284.2948550937799723, -204.6023442560804142 ) ) ;
#62813=CARTESIAN_POINT ( 'NONE',  ( 13.81624004741667555, -278.7687763021331762, -215.4460870757502562 ) ) ;
#62816=CARTESIAN_POINT ( 'NONE',  ( 39.01341242131886133, -274.0424115457452103, -271.1836658468581049 ) ) ;
#62817=CARTESIAN_POINT ( 'NONE',  ( -94.53797134275173164, -277.2585268291529133, -315.9056058551217347 ) ) ;
#62818=CARTESIAN_POINT ( 'NONE',  ( -41.05497484025016774, -296.6198202216361324, -343.9735285365790673 ) ) ;
#62819=CARTESIAN_POINT ( 'NONE',  ( -25.42999032630619638, -279.1209059799435295, -194.6009458692703902 ) ) ;
#62820=CARTESIAN_POINT ( 'NONE',  ( 8.384397823678876094, -295.3499996650740513, -327.6323537776866033 ) ) ;
#62821=CARTESIAN_POINT ( 'NONE',  ( -2.179125175011518589, -295.9116762547243979, -338.3088302090457660 ) ) ;
#62822=CARTESIAN_POINT ( 'NONE',  ( -93.61221286560099486, -297.0449156233469239, -223.8375931050186409 ) ) ;
#62823=CARTESIAN_POINT ( 'NONE',  ( -104.2038043571010206, -293.0027907708559951, -236.2687374149244022 ) ) ;
#62824=CARTESIAN_POINT ( 'NONE',  ( -20.98603584737271532, -286.4231434376322341, -195.1182296114924384 ) ) ;
#62825=CARTESIAN_POINT ( 'NONE',  ( 21.66387114508282963, -274.3393167556122307, -317.9068664561677906 ) ) ;
#62826=CARTESIAN_POINT ( 'NONE',  ( -12.22573453462774395, -288.5676737866609187, -343.2056437545292624 ) ) ;
#62827=CARTESIAN_POINT ( 'NONE',  ( -111.9225191934285988, -280.4921856338110615, -273.4511385940818968 ) ) ;
#62828=CARTESIAN_POINT ( 'NONE',  ( 32.06740669977688185, -286.3015490078142875, -246.9990903011818659 ) ) ;
#62829=CARTESIAN_POINT ( 'NONE',  ( -99.99871612781289798, -289.1094240273531568, -229.0478395601604404 ) ) ;
#62830=CARTESIAN_POINT ( 'NONE',  ( -26.16130516772507875, -127.9538472306148122, -363.7897947155308884 ) ) ;
#62831=CARTESIAN_POINT ( 'NONE',  ( 0.2056653697569757466, -286.0740381543447484, -207.6269091088429946 ) ) ;
#62833=CARTESIAN_POINT ( 'NONE',  ( -44.38564892990635258, -284.0803058584349969, -346.8551583791946769 ) ) ;
#62834=PRODUCT_DEFINITION_FORMATION_WITH_SPECIFIED_SOURCE ( 'ANY', '', #20991, .NOT_KNOWN. ) ;
#62835=CARTESIAN_POINT ( 'NONE',  ( -111.4026152547819208, -289.8651708756594303, -250.1171835078003198 ) ) ;
#62836=CARTESIAN_POINT ( 'NONE',  ( 38.61264438122857712, -283.0750154587286147, -264.2473659342782639 ) ) ;
#62837=CARTESIAN_POINT ( 'NONE',  ( -11.69057627065549099, -281.6943463124954405, -198.2269445011420714 ) ) ;
#62838=CARTESIAN_POINT ( 'NONE',  ( 22.58355914970624312, -281.9665356810629078, -312.0500050509663197 ) ) ;
#62839=CARTESIAN_POINT ( 'NONE',  ( -5.707960850863856628, -276.4682931829216272, -202.3588592535764406 ) ) ;
#62840=CARTESIAN_POINT ( 'NONE',  ( -53.28924607200669072, -295.2510921782077276, -345.7461050271429599 ) ) ;
#62841=CARTESIAN_POINT ( 'NONE',  ( -109.3184322967126860, -288.3144670917659482, -290.3305333247381554 ) ) ;
#62843=CARTESIAN_POINT ( 'NONE',  ( -57.97868720783193908, -296.6995173421065601, -200.0166737305509912 ) ) ;
#62845=CARTESIAN_POINT ( 'NONE',  ( -110.1229130787474730, -286.2693629044856607, -286.0487638383943931 ) ) ;
#62846=CARTESIAN_POINT ( 'NONE',  ( -36.39604677438176594, -293.1434138434801184, -193.6630793353920694 ) ) ;
#62847=CARTESIAN_POINT ( 'NONE',  ( 21.89940733642946569, -282.8021244053456371, -313.2122613418093238 ) ) ;
#62848=CARTESIAN_POINT ( 'NONE',  ( 4.744212798486212357, -273.6639007324630484, -206.0983854134546505 ) ) ;
#62849=CARTESIAN_POINT ( 'NONE',  ( -98.27258978801756939, -291.8305918761275279, -223.4277683630740512 ) ) ;
#62850=CARTESIAN_POINT ( 'NONE',  ( -111.9253693218802965, -282.5186955458379998, -283.9756500099579739 ) ) ;
#62851=CARTESIAN_POINT ( 'NONE',  ( -19.39582449095343009, -292.6100554395524114, -195.4485141377206787 ) ) ;
#62852=CARTESIAN_POINT ( 'NONE',  ( 35.01650413628489389, -287.7510985722426540, -260.1747298294476423 ) ) ;
#62855=CARTESIAN_POINT ( 'NONE',  ( -12.30567835471983251, -92.54755969097151080, -356.2634384826176301 ) ) ;
#62856=CARTESIAN_POINT ( 'NONE',  ( 4.184766045387054767, -284.0238960492750948, -334.4412343949247770 ) ) ;
#62857=CARTESIAN_POINT ( 'NONE',  ( 31.98288692825983404, -290.6237833571634042, -237.0123917617631264 ) ) ;
#62859=CARTESIAN_POINT ( 'NONE',  ( 33.61926898762357752, -280.7150310081751172, -288.8167052985417627 ) ) ;
#62860=CARTESIAN_POINT ( 'NONE',  ( -69.01055622719624694, -277.1240449524029827, -340.5383856355435341 ) ) ;
#62861=CARTESIAN_POINT ( 'NONE',  ( -30.10994822484974875, -282.1438988381503918, -195.8264118833148189 ) ) ;
#62862=CARTESIAN_POINT ( 'NONE',  ( -53.92001451859699301, -170.5180466806795323, -362.3035249365248660 ) ) ;
#62863=CARTESIAN_POINT ( 'NONE',  ( -14.38733816761156703, -278.9186603131959146, -197.4242062396855601 ) ) ;
#62864=CARTESIAN_POINT ( 'NONE',  ( -111.6287668534059065, -282.6729816095882484, -262.5535001505285777 ) ) ;
#62865=CARTESIAN_POINT ( 'NONE',  ( -111.8579010354192462, -274.5902383679150489, -256.3823256773028447 ) ) ;
#62866=CARTESIAN_POINT ( 'NONE',  ( 29.54891209043159961, -294.4395243840719445, -299.7487759107259535 ) ) ;
#62868=CARTESIAN_POINT ( 'NONE',  ( -92.91852436723902997, -289.9176272215531753, -222.2730728309688573 ) ) ;
#62869=CARTESIAN_POINT ( 'NONE',  ( 37.80783614613704913, -276.4085221086491515, -286.7278832686163241 ) ) ;
#62870=CARTESIAN_POINT ( 'NONE',  ( -89.24217123920264783, -273.2962396433483150, -219.0255445617472105 ) ) ;
#62872=CARTESIAN_POINT ( 'NONE',  ( -36.92753951724665740, -272.9775901728838789, -193.6583469963941013 ) ) ;
#62875=CARTESIAN_POINT ( 'NONE',  ( -33.46619183329740821, -284.0819322068512065, -343.5803452570306149 ) ) ;
#62876=CARTESIAN_POINT ( 'NONE',  ( 6.360771649835185393, -284.2281038567240898, -332.5871013470535900 ) ) ;
#62877=CARTESIAN_POINT ( 'NONE',  ( -109.4224865770883923, -283.7821404709110311, -257.3380776408615134 ) ) ;
#62878=CARTESIAN_POINT ( 'NONE',  ( 22.13790592575305993, -273.3465870296930689, -226.6733979653421898 ) ) ;
#62879=CARTESIAN_POINT ( 'NONE',  ( 31.15220526329482453, -283.0349479325320772, -241.7350738599390070 ) ) ;
#62880=CARTESIAN_POINT ( 'NONE',  ( 35.05825435652167243, -273.8523995244961498, -256.6150514733861314 ) ) ;
#62882=CARTESIAN_POINT ( 'NONE',  ( 33.89014266350144311, -276.8601136540028165, -287.7417820347186534 ) ) ;
#62884=CARTESIAN_POINT ( 'NONE',  ( -111.6686336327715026, -279.1099792667473025, -289.8978050649414513 ) ) ;
#62887=CARTESIAN_POINT ( 'NONE',  ( -112.9736449498444273, -286.3452761073405100, -275.6554550595270712 ) ) ;
#62888=CARTESIAN_POINT ( 'NONE',  ( -38.35476239077845406, -294.2623382046859319, -343.5155808153809858 ) ) ;
#62889=CARTESIAN_POINT ( 'NONE',  ( -31.84236128172311098, -288.3331975713170436, -347.1147782188801330 ) ) ;
#62890=CARTESIAN_POINT ( 'NONE',  ( -9.086074484738658086, -284.6666156356701549, -201.9398650835979367 ) ) ;
#62891=CARTESIAN_POINT ( 'NONE',  ( -110.9086457292433323, -283.0838799473302743, -273.6464854542089711 ) ) ;
#62892=CARTESIAN_POINT ( 'NONE',  ( -89.38937110670140385, -288.0374358351659794, -322.9825390787607375 ) ) ;
#62893=CARTESIAN_POINT ( 'NONE',  ( -105.9414742505485805, -286.1038143642189766, -244.2612809240529259 ) ) ;
#62894=CARTESIAN_POINT ( 'NONE',  ( 33.30816297238585122, -273.8799286643911159, -295.6854099585915492 ) ) ;
#62895=CARTESIAN_POINT ( 'NONE',  ( -2.569593827681122544, -284.9040818245816240, -202.5428220803055694 ) ) ;
#62896=CARTESIAN_POINT ( 'NONE',  ( -110.3339370816083402, -298.7736498775735754, -253.1235428115089405 ) ) ;
#62897=CARTESIAN_POINT ( 'NONE',  ( 15.38143230689477114, -286.3095632045445882, -324.0086489772669438 ) ) ;
#62898=CARTESIAN_POINT ( 'NONE',  ( 7.276217091799201953, -281.6183160108930110, -212.2224417748704468 ) ) ;
#62899=CARTESIAN_POINT ( 'NONE',  ( 18.28507042199051469, -290.2562433912549977, -320.9341382708565220 ) ) ;
#62902=CARTESIAN_POINT ( 'NONE',  ( -34.87666172331756087, -296.9415597403174729, -345.8809020549210800 ) ) ;
#62903=CIRCLE ( 'NONE', #15975, 0.5000000000000004441 ) ;
#62904=CARTESIAN_POINT ( 'NONE',  ( -5.908577103291047905, -278.4651481934769777, -202.2518735649484540 ) ) ;
#62905=CARTESIAN_POINT ( 'NONE',  ( -40.61528673981563742, -291.2091670697136010, -193.5792037521810016 ) ) ;
#62906=CARTESIAN_POINT ( 'NONE',  ( -99.41713041296493714, -294.4045521173682687, -310.3681965872725073 ) ) ;
#62907=CARTESIAN_POINT ( 'NONE',  ( -51.90883385042970133, -278.5467815078978333, -198.2740339955405204 ) ) ;
#62908=CARTESIAN_POINT ( 'NONE',  ( -62.49369408153998506, -271.8021710862097962, -200.2990640778067757 ) ) ;
#62909=CARTESIAN_POINT ( 'NONE',  ( 35.39342291899473025, -294.7293772289272624, -259.8328059852659635 ) ) ;
#62910=CARTESIAN_POINT ( 'NONE',  ( 31.95455697924148097, -295.6233781216988064, -236.9535640164627353 ) ) ;
#62911=CARTESIAN_POINT ( 'NONE',  ( -95.03407431894771662, -295.7135370613038390, -220.3393383413759352 ) ) ;
#62912=CARTESIAN_POINT ( 'NONE',  ( 8.260931808884707905, -290.9059231811346535, -209.5140718200036360 ) ) ;
#62913=CARTESIAN_POINT ( 'NONE',  ( -108.3250105716817018, -292.2318142205533036, -250.9512092582315574 ) ) ;
#62915=CARTESIAN_POINT ( 'NONE',  ( -108.5870575165715906, -291.5746558785640445, -253.6721269581376248 ) ) ;
#62918=CARTESIAN_POINT ( 'NONE',  ( -108.0067872313346555, -292.1352898968351042, -240.7899465098449241 ) ) ;
#62919=CARTESIAN_POINT ( 'NONE',  ( 36.38088179767473918, -279.3721047181546169, -254.6984028828678674 ) ) ;
#62920=CARTESIAN_POINT ( 'NONE',  ( 28.73851934338674852, -293.1316699626568720, -239.2191702651877563 ) ) ;
#62921=CARTESIAN_POINT ( 'NONE',  ( -33.91527208777033309, -280.0941422505261471, -193.4373921830085976 ) ) ;
#62922=CARTESIAN_POINT ( 'NONE',  ( -71.73310343550872403, -283.1609349047666342, -339.2303830446265351 ) ) ;
#62923=CARTESIAN_POINT ( 'NONE',  ( -7.510504608907572432, -286.6601309750301425, -339.0468780394057831 ) ) ;
#62924=CARTESIAN_POINT ( 'NONE',  ( -38.93494977148413483, -281.2118977029681446, -344.5919244412208400 ) ) ;
#62927=CARTESIAN_POINT ( 'NONE',  ( 22.34521453128182245, -279.3895684952228180, -222.7989874003200725 ) ) ;
#62928=CARTESIAN_POINT ( 'NONE',  ( 9.632308049755831547, -285.6018915366936994, -209.7398752982981307 ) ) ;
#62930=CARTESIAN_POINT ( 'NONE',  ( 2.657163409574414548, -294.1981345100086287, -208.2801804540858086 ) ) ;
#62931=CARTESIAN_POINT ( 'NONE',  ( 37.05700466529671644, -276.7572307047765321, -252.8847590872648823 ) ) ;
#62932=CARTESIAN_POINT ( 'NONE',  ( -41.86213296151034768, -276.7773636218395268, -343.2548073034763547 ) ) ;
#62933=CARTESIAN_POINT ( 'NONE',  ( -114.3688950888626010, -290.7438982589487750, -268.3568302062585644 ) ) ;
#62934=CARTESIAN_POINT ( 'NONE',  ( -8.609536595199514863, -280.7590582649959288, -340.3006158934864516 ) ) ;
#62935=CARTESIAN_POINT ( 'NONE',  ( 27.36034946782058697, -293.0780598728592850, -304.7776605350622958 ) ) ;
#62936=CARTESIAN_POINT ( 'NONE',  ( -99.97253308030437324, -293.9939406138062168, -311.7149894650987676 ) ) ;
#62939=CARTESIAN_POINT ( 'NONE',  ( -6.009558495371358333, -291.9830887588749420, -204.3451621647675438 ) ) ;
#62941=CARTESIAN_POINT ( 'NONE',  ( 27.36219212280433055, -290.6237833571632905, -239.2376011013261916 ) ) ;
#62942=CARTESIAN_POINT ( 'NONE',  ( -84.05156032424358159, -294.7348872477481905, -331.3461990942407169 ) ) ;
#62943=CARTESIAN_POINT ( 'NONE',  ( -5.442139754822084896, -278.6069473959025231, -201.6390434204160726 ) ) ;
#62944=CARTESIAN_POINT ( 'NONE',  ( 17.98322886151547095, -288.1393186530651178, -217.4410906866914104 ) ) ;
#62945=CARTESIAN_POINT ( 'NONE',  ( -33.23653420753078791, -285.9384604510279928, -197.4268167114228731 ) ) ;
#62946=CARTESIAN_POINT ( 'NONE',  ( -104.8993250691448651, -279.6786411173748661, -299.9282527001880112 ) ) ;
#62947=CARTESIAN_POINT ( 'NONE',  ( -66.72326839700113510, -293.4591052919566323, -338.9801404968505949 ) ) ;
#62948=CARTESIAN_POINT ( 'NONE',  ( -105.7066689261908152, -298.6873665103134954, -242.0026086325144945 ) ) ;
#62949=CARTESIAN_POINT ( 'NONE',  ( -66.97698224585701610, -276.2443920269375326, -337.5093164660243588 ) ) ;
#62952=CARTESIAN_POINT ( 'NONE',  ( -112.5853914706824384, -296.0155619273755292, -286.6132318385991198 ) ) ;
#62953=CARTESIAN_POINT ( 'NONE',  ( -111.7766795392387280, -292.4611241211823085, -271.2260081213711373 ) ) ;
#62955=CARTESIAN_POINT ( 'NONE',  ( 5.911606060737495838, -289.0997892723691507, -329.3567472422961373 ) ) ;
#62958=CARTESIAN_POINT ( 'NONE',  ( 8.415927329374962795, -279.7199359037391559, -208.6585210858092694 ) ) ;
#62959=CARTESIAN_POINT ( 'NONE',  ( -113.6746020047743855, -297.3201015453374794, -261.0551587327499874 ) ) ;
#62960=CARTESIAN_POINT ( 'NONE',  ( -113.1544149194921545, -288.6811845646618622, -271.1911935244992833 ) ) ;
#62961=CARTESIAN_POINT ( 'NONE',  ( -107.7554091008276629, -297.2839048980356438, -239.1221747997875298 ) ) ;
#62962=CARTESIAN_POINT ( 'NONE',  ( 34.08914667304610191, -294.0861079428870539, -285.5776803526617869 ) ) ;
#62966=CARTESIAN_POINT ( 'NONE',  ( -5.894384702698338252, -290.1663095515484656, -339.8864666494469020 ) ) ;
#62967=CARTESIAN_POINT ( 'NONE',  ( -72.08107566293803359, -282.1233781216987495, -198.2974183793908196 ) ) ;
#62968=CARTESIAN_POINT ( 'NONE',  ( 37.44728912312089619, -281.1253883190915417, -288.3035628995652360 ) ) ;
#62969=CARTESIAN_POINT ( 'NONE',  ( -106.2965543353912778, -286.9345090002192364, -241.1545224080606431 ) ) ;
#62970=CARTESIAN_POINT ( 'NONE',  ( 28.20252731901684484, -285.6095947461273568, -230.9835893174585806 ) ) ;
#62971=CARTESIAN_POINT ( 'NONE',  ( -77.52780789517017013, -271.5113161129791024, -207.2334285922567290 ) ) ;
#62972=CARTESIAN_POINT ( 'NONE',  ( -63.84176572078402501, -275.6240890019755057, -200.7839986880234733 ) ) ;
#62973=CARTESIAN_POINT ( 'NONE',  ( -97.74104977539028027, -288.0353022217424837, -313.8724126285737839 ) ) ;
#62974=CARTESIAN_POINT ( 'NONE',  ( -86.27901104557732026, -279.5828220867237519, -328.2695663050141661 ) ) ;
#62976=ORIENTED_EDGE ( 'NONE', *, *, #87763, .T. ) ;
#62977=CARTESIAN_POINT ( 'NONE',  ( 20.51592719969110235, -280.9254442952920385, -225.8268154904255596 ) ) ;
#62978=CARTESIAN_POINT ( 'NONE',  ( 21.41584665055057712, -280.2915751626857173, -226.8493195680522376 ) ) ;
#62979=CARTESIAN_POINT ( 'NONE',  ( 21.50232542350060427, -277.2963200325701223, -319.5431590923438989 ) ) ;
#62980=CARTESIAN_POINT ( 'NONE',  ( -95.59381759742383622, -278.0217602610235872, -220.5946240181123699 ) ) ;
#62981=CARTESIAN_POINT ( 'NONE',  ( 187.5019281953806853, 269.8710585761918423, -138.0480249882951966 ) ) ;
#62982=CARTESIAN_POINT ( 'NONE',  ( -102.5255871153598122, -274.0254342178769775, -229.8163144950540584 ) ) ;
#62984=CARTESIAN_POINT ( 'NONE',  ( -33.39078516767594351, -299.5259680346137543, -193.9494065657861199 ) ) ;
#62985=CARTESIAN_POINT ( 'NONE',  ( -110.4683760289727132, -287.2662352645559167, -253.7030783399848985 ) ) ;
#62988=CARTESIAN_POINT ( 'NONE',  ( 35.58047339840869938, -288.5330178477315144, -262.8389719184933710 ) ) ;
#62989=CARTESIAN_POINT ( 'NONE',  ( 30.50679229513355395, -288.8661463523419570, -236.1477275161182945 ) ) ;
#62990=CARTESIAN_POINT ( 'NONE',  ( -45.38188668910025569, -288.5052955228564429, -343.0195522360081100 ) ) ;
#62991=CARTESIAN_POINT ( 'NONE',  ( -96.22726432595374035, -283.3923128855403206, -319.8993522678615022 ) ) ;
#62992=CARTESIAN_POINT ( 'NONE',  ( -43.80102293886467635, -278.3691711371228621, -196.7935492732414389 ) ) ;
#62993=CARTESIAN_POINT ( 'NONE',  ( 7.657163490996349964, -288.5337548566711234, -211.2541008828198414 ) ) ;
#62994=CARTESIAN_POINT ( 'NONE',  ( 23.14287389781567228, -280.6133122705425080, -312.4600972807643302 ) ) ;
#62995=CARTESIAN_POINT ( 'NONE',  ( -105.7205482372036442, -279.5095117948940810, -297.2976472374737114 ) ) ;
#62996=CARTESIAN_POINT ( 'NONE',  ( -7.476765155910844562, -277.1420140158919025, -337.0400059527298140 ) ) ;
#62998=CARTESIAN_POINT ( 'NONE',  ( -94.40521616531121651, -290.0439362521408952, -219.2556989306164326 ) ) ;
#62999=CARTESIAN_POINT ( 'NONE',  ( -112.8415326572952040, -285.5373813710221498, -255.8035268155682331 ) ) ;
#63000=CARTESIAN_POINT ( 'NONE',  ( -66.54707913852071499, -283.9168772016176376, -341.5551538606963504 ) ) ;
#63001=CARTESIAN_POINT ( 'NONE',  ( 35.68732266494509275, -281.6953566651343408, -268.5814587123384172 ) ) ;
#63004=CARTESIAN_POINT ( 'NONE',  ( -96.31347582957280906, -291.7642537253607316, -317.9487351927022019 ) ) ;
#63005=CARTESIAN_POINT ( 'NONE',  ( -83.95255868565138258, -290.1120748682668591, -209.6253705470738851 ) ) ;
#63006=CARTESIAN_POINT ( 'NONE',  ( 33.81229415644681779, -274.8395173125319388, -287.7493502481726750 ) ) ;
#63007=CARTESIAN_POINT ( 'NONE',  ( -88.54375269322400754, -295.0963862060222596, -327.8055429196993487 ) ) ;
#63008=CARTESIAN_POINT ( 'NONE',  ( -95.65122973878563073, -289.6605476513375379, -225.2977569117147141 ) ) ;
#63009=CARTESIAN_POINT ( 'NONE',  ( -37.01325550997965053, -293.2878102028650460, -344.3863221695962693 ) ) ;
#63010=CARTESIAN_POINT ( 'NONE',  ( -48.10412734459646344, -290.3970666987169125, -343.0161400735657935 ) ) ;
#63011=CARTESIAN_POINT ( 'NONE',  ( 144.7857639756989272, -299.5541904835127980, -195.3611179825600175 ) ) ;
#63012=CARTESIAN_POINT ( 'NONE',  ( -106.5321357785026350, -292.9302466554339617, -241.4183423629412459 ) ) ;
#63013=CARTESIAN_POINT ( 'NONE',  ( 34.54137347435882077, -291.2693564594903251, -248.3872208175358196 ) ) ;
#63014=CARTESIAN_POINT ( 'NONE',  ( 13.53410190626144782, -296.3404442286606582, -325.5364432101684997 ) ) ;
#63015=CARTESIAN_POINT ( 'NONE',  ( -42.70327816994743841, -286.9241369061987257, -197.3096816253706436 ) ) ;
#63016=CARTESIAN_POINT ( 'NONE',  ( -2.787045161349277045, -296.5965519407339457, -337.1144268880131563 ) ) ;
#63017=CARTESIAN_POINT ( 'NONE',  ( 28.49789851870281154, -277.0452721716859514, -233.5993599668678087 ) ) ;
#63018=CARTESIAN_POINT ( 'NONE',  ( 7.881302469686009893, -297.8020023944824857, -193.5285642472007055 ) ) ;
#63019=CARTESIAN_POINT ( 'NONE',  ( 34.87716369859120391, -274.0035260184302501, -286.6177373220539266 ) ) ;
#63020=CARTESIAN_POINT ( 'NONE',  ( 12.28363644438488400, -278.8292342793239982, -214.8756228918846034 ) ) ;
#63021=CARTESIAN_POINT ( 'NONE',  ( -108.3280588312201473, -274.0045668547690525, -251.5095116243433608 ) ) ;
#63022=CARTESIAN_POINT ( 'NONE',  ( -10.53717619024843799, -272.9696853844420161, -198.7497827230926930 ) ) ;
#63023=CARTESIAN_POINT ( 'NONE',  ( -42.41235240578507160, -296.5426295729634489, -343.7754449430537989 ) ) ;
#63026=CARTESIAN_POINT ( 'NONE',  ( -109.0409304586767547, -297.1625973445115960, -284.9775745624945671 ) ) ;
#63028=CARTESIAN_POINT ( 'NONE',  ( -77.28637229139522447, -287.6046118384602437, -334.3190240826729109 ) ) ;
#63029=CARTESIAN_POINT ( 'NONE',  ( -49.95391831840064611, -297.8867250657352770, -198.4588791278499684 ) ) ;
#63030=CARTESIAN_POINT ( 'NONE',  ( 9.810754700973625120, -286.6813891697905774, -209.4871005071713057 ) ) ;
#63031=CARTESIAN_POINT ( 'NONE',  ( -109.8470693738500188, -289.8906024269907675, -296.3787106952124759 ) ) ;
#63032=CARTESIAN_POINT ( 'NONE',  ( -103.8148314366280403, -299.0019721543181959, -234.7576870238316360 ) ) ;
#63033=CARTESIAN_POINT ( 'NONE',  ( 36.11935118030471159, -291.7355669314308102, -284.6265436685044392 ) ) ;
#63034=CARTESIAN_POINT ( 'NONE',  ( 39.54891352599890553, -280.7440604015646386, -269.9413761089698482 ) ) ;
#63035=CARTESIAN_POINT ( 'NONE',  ( 21.31550574532286291, -290.4094976428776249, -223.6242672951989618 ) ) ;
#63036=CARTESIAN_POINT ( 'NONE',  ( -91.87266939285095191, -277.2745298032613164, -218.7952315409555695 ) ) ;
#63037=CARTESIAN_POINT ( 'NONE',  ( 21.48256938208964328, -286.9599158639961161, -314.2778893322750946 ) ) ;
#63039=CARTESIAN_POINT ( 'NONE',  ( -17.98113100053491564, -286.8025241097366234, -342.8731896050754244 ) ) ;
#63040=CARTESIAN_POINT ( 'NONE',  ( -92.45575991057086185, -298.8464650905340250, -221.2807672255001421 ) ) ;
#63041=CARTESIAN_POINT ( 'NONE',  ( 35.91899233989964557, -283.2540110621814051, -292.2568177500588149 ) ) ;
#63042=CARTESIAN_POINT ( 'NONE',  ( -104.3209367327989412, -271.0930668772665513, -235.2753132652601664 ) ) ;
#63043=CARTESIAN_POINT ( 'NONE',  ( 25.13628627644695257, -281.0312801971525687, -232.5073484677236308 ) ) ;
#63044=CARTESIAN_POINT ( 'NONE',  ( -101.5508621032647767, -297.2781296578212391, -227.8378898526343050 ) ) ;
#63045=CARTESIAN_POINT ( 'NONE',  ( 23.52960700504146629, -276.4066530978067817, -228.9856649250569092 ) ) ;
#63046=CARTESIAN_POINT ( 'NONE',  ( 36.09891721298755840, -285.8591459495142431, -288.1861810035260874 ) ) ;
#63048=CARTESIAN_POINT ( 'NONE',  ( 36.18987807317616046, -283.7419359971148083, -285.1295863958147265 ) ) ;
#63049=CARTESIAN_POINT ( 'NONE',  ( -81.24518144970640776, -272.3600777484548985, -211.5887380426867423 ) ) ;
#63052=CARTESIAN_POINT ( 'NONE',  ( 82.64890176555634582, -299.5541904835127980, -195.3611179825600175 ) ) ;
#63053=CARTESIAN_POINT ( 'NONE',  ( -109.9716505721188895, -286.7549320166768894, -253.0799303444032944 ) ) ;
#63055=CARTESIAN_POINT ( 'NONE',  ( 44.71564893372296723, -279.0523547857346784, -270.3937649182068412 ) ) ;
#63056=CARTESIAN_POINT ( 'NONE',  ( -17.40965896147221770, -275.9984474728133819, -344.5694231441364082 ) ) ;
#63057=CARTESIAN_POINT ( 'NONE',  ( 6.015484892702065878, -283.9719618248271331, -329.9502298889095755 ) ) ;
#63058=CARTESIAN_POINT ( 'NONE',  ( 22.11372566371886350, -276.5463265229942067, -226.6404962973884949 ) ) ;
#63059=CARTESIAN_POINT ( 'NONE',  ( -113.2365138387976913, -286.0891424024634944, -261.4963819996870598 ) ) ;
#63060=CARTESIAN_POINT ( 'NONE',  ( -59.08029767950522171, -282.1345941859328832, -340.5185030085810922 ) ) ;
#63061=CARTESIAN_POINT ( 'NONE',  ( 23.72760538252448370, -282.9602990357549857, -226.8233117126235925 ) ) ;
#63062=CARTESIAN_POINT ( 'NONE',  ( -63.55908921140584766, -273.8863641589410918, -197.9618879165280987 ) ) ;
#63063=CARTESIAN_POINT ( 'NONE',  ( 24.36638555847289922, -275.9981441450905209, -316.4166514766521914 ) ) ;
#63064=CARTESIAN_POINT ( 'NONE',  ( -47.97502623523742926, -297.1084677946071224, -344.0900425622648413 ) ) ;
#63067=CARTESIAN_POINT ( 'NONE',  ( -110.4241862647871670, -294.9483128571727661, -250.1861018454835062 ) ) ;
#63068=CARTESIAN_POINT ( 'NONE',  ( 34.68738188461561833, -274.8975026681275722, -258.0474996951396633 ) ) ;
#63069=CARTESIAN_POINT ( 'NONE',  ( -113.7859253652709555, -273.8287563820230162, -264.6711018824900066 ) ) ;
#63070=CARTESIAN_POINT ( 'NONE',  ( -67.98745683035579646, -287.4043267569894056, -202.9904150614670755 ) ) ;
#63071=CARTESIAN_POINT ( 'NONE',  ( -30.63245572179668486, -296.4888931318121195, -346.3722605337579807 ) ) ;
#63072=CARTESIAN_POINT ( 'NONE',  ( 36.31809992813148114, -294.4916979435695907, -249.2837921777557426 ) ) ;
#63073=CARTESIAN_POINT ( 'NONE',  ( -98.03088127986349321, -291.9549833860205013, -314.1429831729067246 ) ) ;
#63074=CARTESIAN_POINT ( 'NONE',  ( -36.97439094717415742, -278.0566052597273483, -195.5286817324358140 ) ) ;
#63075=CARTESIAN_POINT ( 'NONE',  ( -90.51906250471800774, -281.2123537666566335, -218.1969437695659622 ) ) ;
#63076=CARTESIAN_POINT ( 'NONE',  ( -74.03306107362777766, -293.6235409237839349, -335.1303871671878483 ) ) ;
#63077=CARTESIAN_POINT ( 'NONE',  ( -24.71571648141593869, -284.7532668527419446, -345.1197231323229744 ) ) ;
#63078=CARTESIAN_POINT ( 'NONE',  ( -95.19254975189075196, -284.1044808988198156, -225.3129113376041914 ) ) ;
#63079=CARTESIAN_POINT ( 'NONE',  ( 203.7351382603598040, 291.4157354431145563, -82.94369648350118496 ) ) ;
#63081=CARTESIAN_POINT ( 'NONE',  ( -108.1147665232138735, -283.9816324131753618, -288.3405662467736192 ) ) ;
#63084=CARTESIAN_POINT ( 'NONE',  ( 1.947632823567920779, -283.6188862224968830, -336.2234048076468298 ) ) ;
#63085=CARTESIAN_POINT ( 'NONE',  ( -104.4008067951902063, -273.2751936714635690, -241.3337623239234233 ) ) ;
#63086=CARTESIAN_POINT ( 'NONE',  ( -12.81623908733407013, -285.1589429710763852, -197.7903905596899392 ) ) ;
#63087=CARTESIAN_POINT ( 'NONE',  ( 37.75198460200883943, -282.2927762242015319, -254.3684718586702331 ) ) ;
#63089=CARTESIAN_POINT ( 'NONE',  ( -101.5034207699642792, -279.5242982955755338, -311.7610266103919230 ) ) ;
#63090=CARTESIAN_POINT ( 'NONE',  ( -17.02691315267212246, -280.9591996657974846, -196.1949382478952373 ) ) ;
#63091=CARTESIAN_POINT ( 'NONE',  ( -53.28691492658257545, -277.3380690714490129, -200.3538533559491555 ) ) ;
#63092=CARTESIAN_POINT ( 'NONE',  ( 204.3871269384557934, 295.4037104000961449, -68.67796409040960270 ) ) ;
#63094=CARTESIAN_POINT ( 'NONE',  ( -24.30138684413341110, -276.2190463901577573, -196.6198480844160770 ) ) ;
#63095=CARTESIAN_POINT ( 'NONE',  ( 202.8071025886960115, 295.9636416993531611, -68.64508862776258979 ) ) ;
#63096=CARTESIAN_POINT ( 'NONE',  ( -99.34612708073704823, -277.1379002975523917, -228.7086077216202398 ) ) ;
#63097=CARTESIAN_POINT ( 'NONE',  ( 38.42891235670971639, -295.2397248284237321, -264.6350114898483525 ) ) ;
#63098=CARTESIAN_POINT ( 'NONE',  ( -90.48703787331659498, -295.1780869321464706, -320.6283069397197210 ) ) ;
#63099=CARTESIAN_POINT ( 'NONE',  ( -37.78837661708388396, -291.5543535914056861, -193.4239528171910081 ) ) ;
#63101=CARTESIAN_POINT ( 'NONE',  ( -101.1463353411968171, -294.5687360818945990, -312.4993777970919950 ) ) ;
#63102=CARTESIAN_POINT ( 'NONE',  ( 0.5972259697621423724, -284.9664356176119213, -207.0000439995350803 ) ) ;
#63103=CARTESIAN_POINT ( 'NONE',  ( 2.890354310803937121, -294.4583801239031686, -207.9123580034386407 ) ) ;
#63104=CARTESIAN_POINT ( 'NONE',  ( 30.93717668364962847, -286.5999599355418468, -297.6872333717078050 ) ) ;
#63105=CARTESIAN_POINT ( 'NONE',  ( -94.65916787433052093, -285.2214069291394480, -316.3806026674670306 ) ) ;
#63106=ORIENTED_EDGE ( 'NONE', *, *, #60023, .F. ) ;
#63107=CARTESIAN_POINT ( 'NONE',  ( -61.62554693549186169, -292.6855577214944333, -197.4826398874059521 ) ) ;
#63108=CARTESIAN_POINT ( 'NONE',  ( 33.71146714199196737, -282.2694403430483590, -287.4271767031661966 ) ) ;
#63109=CARTESIAN_POINT ( 'NONE',  ( -113.5497597816783042, -295.2494269696082370, -278.1290238641061592 ) ) ;
#63110=CARTESIAN_POINT ( 'NONE',  ( -105.8647498219482799, -291.8048447638614675, -235.4766814274685771 ) ) ;
#63111=CARTESIAN_POINT ( 'NONE',  ( -91.55071776032434627, -290.2911720534075357, -325.0337612924163295 ) ) ;
#63112=CARTESIAN_POINT ( 'NONE',  ( 14.08488714284487209, -288.4717125818122554, -322.1714077536313994 ) ) ;
#63115=CARTESIAN_POINT ( 'NONE',  ( -67.70899896146165986, -297.3068286217032892, -339.7738880202303449 ) ) ;
#63116=CARTESIAN_POINT ( 'NONE',  ( -113.2832330124605846, -295.3538313999151228, -261.0776996753071444 ) ) ;
#63118=CARTESIAN_POINT ( 'NONE',  ( 9.436009348219009496, -279.7721314182165315, -213.9456066480778134 ) ) ;
#63119=CARTESIAN_POINT ( 'NONE',  ( 39.31865375809432805, -275.1416111320269238, -276.8969457918657326 ) ) ;
#63120=CARTESIAN_POINT ( 'NONE',  ( -94.98162655975804114, -295.6743921351554150, -224.4443820820378335 ) ) ;
#63121=CARTESIAN_POINT ( 'NONE',  ( -48.77509254653654125, -279.0595779434141264, -343.7628323835089645 ) ) ;
#63122=CARTESIAN_POINT ( 'NONE',  ( 34.05443350719821183, -273.4252093852364283, -249.8435697581917907 ) ) ;
#63123=CARTESIAN_POINT ( 'NONE',  ( -100.5003757326617375, -297.2450203460318789, -307.8524960164338040 ) ) ;
#63124=CARTESIAN_POINT ( 'NONE',  ( -84.28326906784921846, -298.4686000627070825, -213.9857250814623342 ) ) ;
#63126=CARTESIAN_POINT ( 'NONE',  ( -83.68236812177651984, -297.2758586651191308, -330.9171585209741693 ) ) ;
#63127=CARTESIAN_POINT ( 'NONE',  ( -35.84733324182673186, -296.0706611987501446, -195.1949506821764828 ) ) ;
#63128=CARTESIAN_POINT ( 'NONE',  ( -36.21286596702780258, -292.7180537408303280, -197.2554067769167148 ) ) ;
#63129=CARTESIAN_POINT ( 'NONE',  ( -76.35955921404796243, -274.3475378469351540, -204.1047283533753216 ) ) ;
#63130=CARTESIAN_POINT ( 'NONE',  ( -102.9265355052720707, -289.5779091805952703, -236.8716692833707214 ) ) ;
#63132=CARTESIAN_POINT ( 'NONE',  ( -64.88391296044297007, -274.1942506620181916, -198.5071671305449854 ) ) ;
#63133=CARTESIAN_POINT ( 'NONE',  ( -104.7833613082437836, -297.2607361762896971, -242.3663001772050052 ) ) ;
#63134=CARTESIAN_POINT ( 'NONE',  ( 11.89794985329147714, -282.7123680097561191, -213.3184701681800846 ) ) ;
#63135=CARTESIAN_POINT ( 'NONE',  ( 34.12086354064076232, -280.5850996415467762, -297.6814449517692651 ) ) ;
#63136=CARTESIAN_POINT ( 'NONE',  ( -5.334775114619859870, -275.9905264373508089, -340.2815694842814764 ) ) ;
#63137=CARTESIAN_POINT ( 'NONE',  ( 38.39009685180050724, -279.8395848113973443, -261.4638217592255955 ) ) ;
#63138=CARTESIAN_POINT ( 'NONE',  ( 31.50423271860621455, -279.1578583481900182, -240.1905039001952105 ) ) ;
#63140=CARTESIAN_POINT ( 'NONE',  ( -48.95063505970350803, -272.4762336020547195, -197.6417438854277577 ) ) ;
#63141=CARTESIAN_POINT ( 'NONE',  ( -110.7929881235739202, -280.7477983140753963, -255.1360513273831998 ) ) ;
#63144=CARTESIAN_POINT ( 'NONE',  ( -113.0653769905977981, -271.0595318834638761, -261.8543455666935529 ) ) ;
#63145=CARTESIAN_POINT ( 'NONE',  ( -68.32876473972254416, -291.6562548435997542, -199.8570225637258204 ) ) ;
#63146=CARTESIAN_POINT ( 'NONE',  ( -38.49076503620204193, -279.0666862774626793, -345.5190056618538392 ) ) ;
#63147=CARTESIAN_POINT ( 'NONE',  ( 8.574916681755698988, -272.6810440905719588, -211.0596429048015921 ) ) ;
#63149=CARTESIAN_POINT ( 'NONE',  ( 0.1750251051061615104, -284.4769181089097856, -335.9642490314248562 ) ) ;
#63151=CARTESIAN_POINT ( 'NONE',  ( 5.515036019150874047, -284.6318351268753872, -208.7496893978193384 ) ) ;
#63153=CARTESIAN_POINT ( 'NONE',  ( -35.65680163459835939, -293.8255016288889578, -343.7514147180479540 ) ) ;
#63154=CARTESIAN_POINT ( 'NONE',  ( 36.91660228816733280, -285.6650103968020744, -268.3014338869509743 ) ) ;
#63156=CARTESIAN_POINT ( 'NONE',  ( -42.55345161240357754, -293.1177497459933079, -345.1798208316198497 ) ) ;
#63157=CARTESIAN_POINT ( 'NONE',  ( -12.90723809123782040, -284.8439475063588020, -198.0723580218308939 ) ) ;
#63158=CARTESIAN_POINT ( 'NONE',  ( -81.78572700359976011, -281.0358703315853290, -211.3803096988781647 ) ) ;
#63159=CARTESIAN_POINT ( 'NONE',  ( -12.84528491914726622, -287.5687060532595183, -197.7805809229789418 ) ) ;
#63160=CARTESIAN_POINT ( 'NONE',  ( 23.43099795397060703, -280.4072464380158749, -315.9752954267714813 ) ) ;
#63161=CARTESIAN_POINT ( 'NONE',  ( 31.39940023454654394, -287.8792892662658005, -294.9306340733404568 ) ) ;
#63162=CARTESIAN_POINT ( 'NONE',  ( -87.94890572964960995, -280.7532821244134311, -216.8651642317157098 ) ) ;
#63163=CARTESIAN_POINT ( 'NONE',  ( -5.497429458520055157, -281.2849928933199521, -204.4934919960515458 ) ) ;
#63165=CARTESIAN_POINT ( 'NONE',  ( -5.492548306803323399, -288.4489274860670776, -202.0673530014701669 ) ) ;
#63167=CARTESIAN_POINT ( 'NONE',  ( -51.79853284000595437, -297.7055434284678199, -194.6760974100936892 ) ) ;
#63168=CARTESIAN_POINT ( 'NONE',  ( -111.7603470849426941, -292.4490297384436417, -276.7962479067879258 ) ) ;
#63170=CARTESIAN_POINT ( 'NONE',  ( 36.60358173371528068, -296.4805209788416391, -305.9350535429201159 ) ) ;
#63172=CARTESIAN_POINT ( 'NONE',  ( 20.45784610560596306, -272.8899438396260280, -222.3065564363317037 ) ) ;
#63174=CARTESIAN_POINT ( 'NONE',  ( -32.08822024938798023, -293.3868272624400788, -346.3929257053404172 ) ) ;
#63175=CARTESIAN_POINT ( 'NONE',  ( -110.2898752900783705, -271.9727075963631933, -264.8975838380630989 ) ) ;
#63176=CARTESIAN_POINT ( 'NONE',  ( -5.475261845078676970, -290.1452296353871816, -336.8083742534934686 ) ) ;
#63177=CARTESIAN_POINT ( 'NONE',  ( 35.70725670043358235, -283.4672456671130476, -282.2701028520872342 ) ) ;
#63178=CARTESIAN_POINT ( 'NONE',  ( -107.1853551753745535, -291.5773910833514151, -301.4826362517486018 ) ) ;
#63179=CARTESIAN_POINT ( 'NONE',  ( -112.1612496465735376, -292.0691920121191743, -254.3200924198557686 ) ) ;
#63180=CARTESIAN_POINT ( 'NONE',  ( -96.55125785631663859, -287.1838143138775195, -224.3051723028688968 ) ) ;
#63181=CARTESIAN_POINT ( 'NONE',  ( -69.96430761824885280, -279.8009722192398385, -200.5988576831022669 ) ) ;
#63182=CARTESIAN_POINT ( 'NONE',  ( -112.9264217661186223, -294.6059352114793910, -272.4059589295201249 ) ) ;
#63183=CARTESIAN_POINT ( 'NONE',  ( 24.25382670642989069, -282.0004499634582089, -316.5670816507339396 ) ) ;
#63184=CARTESIAN_POINT ( 'NONE',  ( -1.140638441075009890, -276.3982786762053934, -205.5364679814612145 ) ) ;
#63185=EDGE_CURVE ( 'NONE', #75524, #64758, #32339, .T. ) ;
#63186=CARTESIAN_POINT ( 'NONE',  ( -95.99890600148557951, -299.6948066931273615, -223.6242672951989618 ) ) ;
#63187=CARTESIAN_POINT ( 'NONE',  ( 38.69317628720677504, -273.8024309066653927, -271.1833478625718499 ) ) ;
#63189=CARTESIAN_POINT ( 'NONE',  ( 32.28805627210257256, -281.3549154146036244, -292.6546803726682242 ) ) ;
#63190=CARTESIAN_POINT ( 'NONE',  ( -107.2076195978872306, -279.3524840613571314, -301.9029006145521521 ) ) ;
#63191=CARTESIAN_POINT ( 'NONE',  ( -93.73870262587062996, -284.3228560490567247, -218.2044578175995753 ) ) ;
#63192=CARTESIAN_POINT ( 'NONE',  ( -36.21285092549082663, -293.8266023443379709, -196.3437403653989293 ) ) ;
#63193=CARTESIAN_POINT ( 'NONE',  ( -78.42753274434281252, -275.1091337855381767, -206.1863973163608819 ) ) ;
#63194=CARTESIAN_POINT ( 'NONE',  ( -60.73635742049441433, -275.0701293798153984, -197.4636245745144265 ) ) ;
#63196=CARTESIAN_POINT ( 'NONE',  ( -1.472081416084617622, -276.3960717918301384, -333.9979572841067466 ) ) ;
#63197=CARTESIAN_POINT ( 'NONE',  ( -71.75168969512166939, -297.5080764983356403, -336.8282998311944993 ) ) ;
#63198=CARTESIAN_POINT ( 'NONE',  ( -27.57261772641772524, -284.1763831357010304, -196.1681705154648512 ) ) ;
#63199=CARTESIAN_POINT ( 'NONE',  ( -34.95681520275245902, -291.7480253732489928, -193.4060674126369292 ) ) ;
#63200=CARTESIAN_POINT ( 'NONE',  ( 22.00422952914819064, -272.9493759197994223, -225.0641665144460433 ) ) ;
#63201=CARTESIAN_POINT ( 'NONE',  ( 19.98464413268053619, -289.8387149093874200, -320.5816847339579567 ) ) ;
#63202=CARTESIAN_POINT ( 'NONE',  ( -110.6766662959683885, -289.4977101895710803, -268.4399982533130924 ) ) ;
#63204=CARTESIAN_POINT ( 'NONE',  ( 10.76203714416920398, -291.2766798812465368, -210.9243793734091241 ) ) ;
#63205=CARTESIAN_POINT ( 'NONE',  ( -101.6637814664811259, -289.7463750275625216, -305.0335967805089012 ) ) ;
#63207=CARTESIAN_POINT ( 'NONE',  ( 28.42635435392962506, -288.1141349376257494, -230.8118584029870703 ) ) ;
#63208=CARTESIAN_POINT ( 'NONE',  ( -108.3112203614117846, -279.1121394554951394, -253.1734862457694533 ) ) ;
#63209=CARTESIAN_POINT ( 'NONE',  ( -86.20896796138724483, -294.6323435329302924, -329.4668084310036988 ) ) ;
#63210=CARTESIAN_POINT ( 'NONE',  ( -32.32136991245290858, -286.7652765054399993, -193.6139540210300822 ) ) ;
#63211=CARTESIAN_POINT ( 'NONE',  ( -76.09974660554641446, -285.8827376696555120, -203.7898980279237549 ) ) ;
#63212=CARTESIAN_POINT ( 'NONE',  ( -10.96417174173520692, -283.0319818911924585, -338.5051956362725036 ) ) ;
#63213=CARTESIAN_POINT ( 'NONE',  ( 138.8680847268318814, 180.6334471161891031, -241.4751441910937899 ) ) ;
#63214=CARTESIAN_POINT ( 'NONE',  ( -114.3093312043316132, -271.9319807694569135, -283.9828466565109011 ) ) ;
#63215=CARTESIAN_POINT ( 'NONE',  ( 183.5144294471984381, 261.3764885010062926, -151.1767051898502530 ) ) ;
#63216=CARTESIAN_POINT ( 'NONE',  ( 23.93431497806644614, -274.1966492604556151, -230.3879807570918103 ) ) ;
#63217=CARTESIAN_POINT ( 'NONE',  ( 35.91006722011604779, -274.5247815569367731, -274.3430696287165347 ) ) ;
#63218=CARTESIAN_POINT ( 'NONE',  ( -111.5343403596023819, -295.8044288841543903, -290.7321522920910297 ) ) ;
#63219=CARTESIAN_POINT ( 'NONE',  ( 85.54234477158686900, 81.19049204599852487, -299.1564525335649591 ) ) ;
#63220=CARTESIAN_POINT ( 'NONE',  ( 37.73804855772906564, -274.0518521039967368, -255.6529701949339426 ) ) ;
#63221=CARTESIAN_POINT ( 'NONE',  ( -91.88425395836236476, -275.0206243463375131, -220.3115213371761456 ) ) ;
#63222=CARTESIAN_POINT ( 'NONE',  ( -91.91241638468210340, -292.3295968127715696, -221.3906983321252540 ) ) ;
#63224=CARTESIAN_POINT ( 'NONE',  ( -103.6526159665097424, -297.9993407255161628, -231.5822784496067470 ) ) ;
#63225=CARTESIAN_POINT ( 'NONE',  ( 35.51378855602177254, -288.1251559077391562, -276.4802535409087909 ) ) ;
#63226=CARTESIAN_POINT ( 'NONE',  ( -68.15202833535775540, -296.2494162280391379, -340.7520442207594442 ) ) ;
#63227=CARTESIAN_POINT ( 'NONE',  ( -101.5734321378067335, -296.4860463053695980, -312.8108698787508501 ) ) ;
#63228=CARTESIAN_POINT ( 'NONE',  ( 8.847199111232466606, -292.8725799752006083, -213.7660430709252353 ) ) ;
#63230=CARTESIAN_POINT ( 'NONE',  ( 9.649993932451877754, -278.3319237031839180, -329.5979980628904400 ) ) ;
#63233=CARTESIAN_POINT ( 'NONE',  ( 21.92731382997954981, -280.3998111506041937, -221.3028782268150962 ) ) ;
#63235=CARTESIAN_POINT ( 'NONE',  ( 11.91479219664280720, -277.2890571715314536, -324.6259421384361872 ) ) ;
#63236=CARTESIAN_POINT ( 'NONE',  ( 24.48912554410425813, -276.7191217165149055, -226.1696133046375792 ) ) ;
#63237=CARTESIAN_POINT ( 'NONE',  ( -112.4421988741684402, -276.4854099179709692, -277.1571048728020514 ) ) ;
#63238=CARTESIAN_POINT ( 'NONE',  ( -77.57498951706452317, -298.1481362308763892, -209.2660732051698176 ) ) ;
#63239=CARTESIAN_POINT ( 'NONE',  ( -100.6828221755220909, -294.6150959388896808, -307.9218366813141756 ) ) ;
#63241=CARTESIAN_POINT ( 'NONE',  ( 22.82326365675837820, -281.4017117710948241, -222.3849455507653090 ) ) ;
#63242=CARTESIAN_POINT ( 'NONE',  ( 33.89373311509346109, -275.9300352735922388, -286.3714315939866424 ) ) ;
#63243=CARTESIAN_POINT ( 'NONE',  ( 13.92890161770685076, -285.4381813583173084, -213.5042571678424963 ) ) ;
#63244=CARTESIAN_POINT ( 'NONE',  ( -40.39199204732053516, -300.0141807766151487, -195.2054793147930525 ) ) ;
#63246=CARTESIAN_POINT ( 'NONE',  ( 20.47453412858477506, -286.1192738877761030, -225.5293794050041924 ) ) ;
#63247=CARTESIAN_POINT ( 'NONE',  ( 20.48154518866151363, -279.1482848145506068, -224.1610496080544124 ) ) ;
#63248=CARTESIAN_POINT ( 'NONE',  ( -74.79012999345189883, -278.1182157286625056, -206.9543895945637644 ) ) ;
#63249=CARTESIAN_POINT ( 'NONE',  ( -51.31165164250147370, -281.3118382834701947, -343.5311176431419540 ) ) ;
#63250=CARTESIAN_POINT ( 'NONE',  ( -5.285663586863666552, -288.4740437397809956, -202.5430161413130747 ) ) ;
#63251=CARTESIAN_POINT ( 'NONE',  ( -26.95021117837024605, -278.1221545454647526, -343.0188599066872825 ) ) ;
#63253=CARTESIAN_POINT ( 'NONE',  ( 22.36712787761467780, -294.9310972204266363, -224.9543510085378557 ) ) ;
#63254=CARTESIAN_POINT ( 'NONE',  ( -111.1956788631972870, -276.5647775228716228, -288.2920306373241033 ) ) ;
#63255=CARTESIAN_POINT ( 'NONE',  ( -59.21761157775852524, -277.9943410688059089, -340.1130868881748484 ) ) ;
#63256=CARTESIAN_POINT ( 'NONE',  ( 20.22282853303963535, -284.2189616330234117, -318.6969584108889535 ) ) ;
#63258=CARTESIAN_POINT ( 'NONE',  ( -107.4530336370362562, -292.1079338968769434, -298.5340679407805169 ) ) ;
#63259=CARTESIAN_POINT ( 'NONE',  ( -112.3178643632237339, -294.5950691873683809, -267.0058100862269725 ) ) ;
#63260=CARTESIAN_POINT ( 'NONE',  ( -35.14259250810531654, -285.2762442845022974, -193.5409534053348750 ) ) ;
#63262=CARTESIAN_POINT ( 'NONE',  ( 29.54175329825874030, -273.8275906543187261, -239.7773650165581500 ) ) ;
#63263=CARTESIAN_POINT ( 'NONE',  ( 22.81941209189212927, -291.0932141143767353, -226.8480447967785381 ) ) ;
#63266=CARTESIAN_POINT ( 'NONE',  ( -110.9587438908396422, -289.2863944448677671, -250.2307816561519758 ) ) ;
#63267=CARTESIAN_POINT ( 'NONE',  ( -95.73708873633613337, -285.5235509007023893, -315.5084392600292063 ) ) ;
#63268=CARTESIAN_POINT ( 'NONE',  ( -21.17738660665003891, -284.4966322767228917, -196.1136333135789869 ) ) ;
#63269=CARTESIAN_POINT ( 'NONE',  ( -107.0966143826628354, -286.2882375635215908, -246.7573178097935340 ) ) ;
#63270=CARTESIAN_POINT ( 'NONE',  ( -83.75819036978028009, -286.1991106314869739, -213.7434415420709115 ) ) ;
#63271=CARTESIAN_POINT ( 'NONE',  ( -105.7774696973465609, -292.9457699474629067, -238.6938416093715603 ) ) ;
#63272=CARTESIAN_POINT ( 'NONE',  ( 36.54258831923565509, -273.4295390553292009, -254.4750028838569449 ) ) ;
#63273=CARTESIAN_POINT ( 'NONE',  ( -17.35929706935331041, -277.1343783495568687, -344.7012004377090193 ) ) ;
#63274=CARTESIAN_POINT ( 'NONE',  ( -108.1162850536406239, -288.9747752233414531, -243.7494825035878989 ) ) ;
#63275=CARTESIAN_POINT ( 'NONE',  ( -82.23885752248339998, -279.4580821340770171, -207.8051809509536838 ) ) ;
#63276=CARTESIAN_POINT ( 'NONE',  ( -70.43102110461339294, -297.4704528193520332, -337.2710846843863237 ) ) ;
#63279=CARTESIAN_POINT ( 'NONE',  ( -109.6754384916872880, -283.4082788649991471, -257.2875719025667536 ) ) ;
#63280=CARTESIAN_POINT ( 'NONE',  ( -31.21115950989508292, -278.1293027334774592, -195.5607684447492716 ) ) ;
#63282=CARTESIAN_POINT ( 'NONE',  ( 34.07968044430916166, -273.6890826553030820, -243.4967522051013020 ) ) ;
#63283=CARTESIAN_POINT ( 'NONE',  ( -109.1449719022743778, -277.7191543809244649, -284.1452712682504398 ) ) ;
#63284=CARTESIAN_POINT ( 'NONE',  ( -36.97281847377762887, -296.5675419774173633, -344.0660731612117047 ) ) ;
#63285=CARTESIAN_POINT ( 'NONE',  ( 39.21963152212485682, -280.5389356741616780, -275.6533220712422008 ) ) ;
#63286=CARTESIAN_POINT ( 'NONE',  ( 19.02183748762764282, -295.1544676015564619, -317.1217860302025429 ) ) ;
#63287=CARTESIAN_POINT ( 'NONE',  ( -102.6856361244626754, -297.3443446626416744, -310.1539351794719437 ) ) ;
#63288=CARTESIAN_POINT ( 'NONE',  ( -39.16620042462899676, -297.8619763040144903, -197.3715125946057469 ) ) ;
#63289=CARTESIAN_POINT ( 'NONE',  ( -112.3366323615187525, -292.5411176586992497, -271.2333478531952551 ) ) ;
#63290=CARTESIAN_POINT ( 'NONE',  ( -107.9269797263946629, -285.1125860053548422, -239.4590038071630431 ) ) ;
#63291=CARTESIAN_POINT ( 'NONE',  ( 17.98476997060967975, -274.4092843453402111, -322.1229493548431719 ) ) ;
#63292=CARTESIAN_POINT ( 'NONE',  ( 20.57149925643157218, -288.0721919372417119, -321.1260430685949814 ) ) ;
#63293=CARTESIAN_POINT ( 'NONE',  ( -62.89519318174656348, -281.6978572709766127, -200.1719240426389206 ) ) ;
#63295=CARTESIAN_POINT ( 'NONE',  ( -103.6935821020003630, -284.0295633711314167, -239.2435851917049092 ) ) ;
#63296=AXIS2_PLACEMENT_3D ( 'NONE', #8528, #37407, #66316 ) ;
#63297=CARTESIAN_POINT ( 'NONE',  ( -7.733544505421187765, -286.6639937694782816, -339.2833144905030736 ) ) ;
#63298=CARTESIAN_POINT ( 'NONE',  ( 26.40820234725076787, -24.66803830325296687, -341.1985388896944755 ) ) ;
#63299=CARTESIAN_POINT ( 'NONE',  ( -41.32001614970636894, -285.5084000093574446, -197.3954635197628704 ) ) ;
#63301=CARTESIAN_POINT ( 'NONE',  ( -41.54423160417324823, -284.0449741152323782, -347.0628703967219622 ) ) ;
#63302=CARTESIAN_POINT ( 'NONE',  ( -101.4807494939215502, -290.1681617457197717, -228.0875275019855337 ) ) ;
#63303=CARTESIAN_POINT ( 'NONE',  ( -109.8985848374399126, -279.8545586158737137, -293.8104415641644778 ) ) ;
#63304=CARTESIAN_POINT ( 'NONE',  ( -100.0516267721233845, -279.2842137432617733, -314.1876324846426769 ) ) ;
#63305=CARTESIAN_POINT ( 'NONE',  ( 11.30739951486635242, -280.5824260019657572, -215.9344231681857025 ) ) ;
#63306=CARTESIAN_POINT ( 'NONE',  ( 37.09421864241076605, -277.6755328977007480, -279.9576504304097284 ) ) ;
#63307=CARTESIAN_POINT ( 'NONE',  ( -56.07028341321783671, -295.2869415952472423, -345.0487352168224788 ) ) ;
#63308=CARTESIAN_POINT ( 'NONE',  ( -108.5281749271665888, -288.2791341774243961, -292.9896135880377415 ) ) ;
#63309=CARTESIAN_POINT ( 'NONE',  ( -108.2721384043396995, -295.2283654606972050, -288.9337183668135935 ) ) ;
#63312=CARTESIAN_POINT ( 'NONE',  ( -68.36259239206556515, -285.3830385236655047, -338.0295629498184553 ) ) ;
#63313=CARTESIAN_POINT ( 'NONE',  ( -107.4784947900113821, -296.4875622568389417, -250.0407459051728267 ) ) ;
#63314=CARTESIAN_POINT ( 'NONE',  ( -25.08444572857407096, -293.2846291714917015, -194.6560836479893339 ) ) ;
#63315=CARTESIAN_POINT ( 'NONE',  ( -84.92185123040701455, -284.3806409966656474, -325.8590628898555224 ) ) ;
#63316=CARTESIAN_POINT ( 'NONE',  ( -18.59579272537223815, -273.3465019727900653, -195.8655987189355869 ) ) ;
#63317=CARTESIAN_POINT ( 'NONE',  ( -79.54541412990505478, -292.1499025450798968, -206.0155880775002686 ) ) ;
#63318=CARTESIAN_POINT ( 'NONE',  ( -91.01103837213831582, -283.4393515043308298, -216.8830139408525781 ) ) ;
#63319=CARTESIAN_POINT ( 'NONE',  ( -108.3492679745883720, -291.2636356959866930, -240.6345372850109925 ) ) ;
#63320=CARTESIAN_POINT ( 'NONE',  ( 35.57348053269802080, -287.8223972295223803, -265.5810910896143469 ) ) ;
#63323=CARTESIAN_POINT ( 'NONE',  ( -21.51142200380889946, -109.0746302473303331, -358.9104106151312408 ) ) ;
#63324=CARTESIAN_POINT ( 'NONE',  ( -35.89277258145762772, -284.5544389133588652, -346.6670282107009484 ) ) ;
#63325=CARTESIAN_POINT ( 'NONE',  ( 10.59707575819633618, -291.9094976428776818, -330.5268031993606428 ) ) ;
#63327=CARTESIAN_POINT ( 'NONE',  ( 1.252402303661884098, -281.4442099325958679, -332.7479206258836939 ) ) ;
#63328=CARTESIAN_POINT ( 'NONE',  ( -54.13077262984366911, -276.9286405235873190, -345.5414474655901245 ) ) ;
#63329=CARTESIAN_POINT ( 'NONE',  ( -106.9643909474264518, -280.1943879425912769, -297.7966669535657616 ) ) ;
#63330=CARTESIAN_POINT ( 'NONE',  ( 181.5289669338484657, 251.5006589549888645, -165.3271292094310070 ) ) ;
#63331=CARTESIAN_POINT ( 'NONE',  ( 27.36214648389219306, -279.5894814000602651, -229.6168920535202744 ) ) ;
#63332=CARTESIAN_POINT ( 'NONE',  ( -110.3336466543562580, -282.3699478421068534, -286.0431409718472651 ) ) ;
#63333=CARTESIAN_POINT ( 'NONE',  ( -97.45882870465375447, -297.6836258872466487, -316.8358946755942611 ) ) ;
#63334=CARTESIAN_POINT ( 'NONE',  ( 34.54259340403847034, -293.8714098260960554, -257.2287812982983723 ) ) ;
#63336=CARTESIAN_POINT ( 'NONE',  ( -104.5051629824076116, -288.8365008741224642, -300.3249704701875089 ) ) ;
#63337=CARTESIAN_POINT ( 'NONE',  ( 25.98765919217384734, -276.7812294726693381, -314.0733021426435698 ) ) ;
#63338=CARTESIAN_POINT ( 'NONE',  ( -87.33330285485418187, -273.3318000072327436, -217.0956709510115274 ) ) ;
#63340=CARTESIAN_POINT ( 'NONE',  ( -13.14692271601287032, -273.2796180865968836, -197.5867732229094429 ) ) ;
#63344=CARTESIAN_POINT ( 'NONE',  ( -4.677132606053719499, -283.6910173250950038, -335.9907766988711728 ) ) ;
#63345=CARTESIAN_POINT ( 'NONE',  ( -5.390743042716076516, -282.2269186829847172, -201.4183130037586977 ) ) ;
#63346=CARTESIAN_POINT ( 'NONE',  ( -91.84815931963028390, -282.9129456252104546, -319.2927134845928663 ) ) ;
#63347=CARTESIAN_POINT ( 'NONE',  ( -8.793868743443603364, -282.2900916284773984, -201.8345771032478240 ) ) ;
#63348=CARTESIAN_POINT ( 'NONE',  ( 24.38471855504198160, -273.4794755556297901, -230.1049757329376462 ) ) ;
#63353=CARTESIAN_POINT ( 'NONE',  ( -112.3245841357175294, -279.1446233611774801, -287.1458112260974644 ) ) ;
#63357=CARTESIAN_POINT ( 'NONE',  ( -32.41085433867187504, -287.9740840468297165, -194.7439814509482403 ) ) ;
#63358=CARTESIAN_POINT ( 'NONE',  ( 0.0002403523676656696027, -291.7601370730342865, -207.4470400019629892 ) ) ;
#63359=CARTESIAN_POINT ( 'NONE',  ( -43.18283780114209947, -288.4726747380678944, -347.0370196550280184 ) ) ;
#63360=CARTESIAN_POINT ( 'NONE',  ( -67.94653331856557088, -283.8846137902221471, -202.9718146672726959 ) ) ;
#63361=CARTESIAN_POINT ( 'NONE',  ( -96.22661192625950832, -283.7414727544141329, -226.2256211456656558 ) ) ;
#63362=CARTESIAN_POINT ( 'NONE',  ( -56.34712896225217804, -287.5401149642161158, -341.9459940440991659 ) ) ;
#63364=CARTESIAN_POINT ( 'NONE',  ( -103.3631639362055097, -285.3240595082319260, -302.5448580271842047 ) ) ;
#63365=CARTESIAN_POINT ( 'NONE',  ( 34.95083735305195205, -273.8093906626360763, -290.3786626950142704 ) ) ;
#63366=CARTESIAN_POINT ( 'NONE',  ( 17.78695433068271115, -285.2244864174737700, -217.6801330819846783 ) ) ;
#63367=CARTESIAN_POINT ( 'NONE',  ( -90.24334274061806127, -299.3040049424387234, -217.1970619252629433 ) ) ;
#63368=CARTESIAN_POINT ( 'NONE',  ( -84.34615385057271908, -283.4068543128089459, -211.7044069113624403 ) ) ;
#63369=CARTESIAN_POINT ( 'NONE',  ( 9.417588190318248564, -281.6543325051471243, -213.9303381918627451 ) ) ;
#63370=CARTESIAN_POINT ( 'NONE',  ( 34.21057718990975616, -289.8489573500260121, -293.3893623157172783 ) ) ;
#63373=CARTESIAN_POINT ( 'NONE',  ( -1.369764346864409177, -296.4991389612242187, -336.8237069303060593 ) ) ;
#63374=CARTESIAN_POINT ( 'NONE',  ( -36.97363010064713507, -278.0566052562255663, -195.3620168015945069 ) ) ;
#63375=CARTESIAN_POINT ( 'NONE',  ( -112.1079507480223185, -289.5264802661381509, -288.1421918639035766 ) ) ;
#63376=CARTESIAN_POINT ( 'NONE',  ( 1.979022500949452867, -292.9166040905300861, -332.8741832534555556 ) ) ;
#63377=CARTESIAN_POINT ( 'NONE',  ( -6.547601964989245182, -279.1500236574109977, -203.6168238788341682 ) ) ;
#63378=CARTESIAN_POINT ( 'NONE',  ( -41.92126853163554756, -296.1334074908899083, -196.2673055922932690 ) ) ;
#63379=CARTESIAN_POINT ( 'NONE',  ( 17.09224104264845678, -294.1638216175812772, -220.9084719378967634 ) ) ;
#63380=CARTESIAN_POINT ( 'NONE',  ( 21.27581636871892101, -289.4090924074130839, -223.5744983911110353 ) ) ;
#63381=CARTESIAN_POINT ( 'NONE',  ( -97.67376968805652382, -295.6616800873560464, -223.6201368145549964 ) ) ;
#63382=CARTESIAN_POINT ( 'NONE',  ( -31.79106778512614540, -290.5812147842836453, -344.0032664663007154 ) ) ;
#63383=CARTESIAN_POINT ( 'NONE',  ( 36.10892248153815842, -291.5444706346461885, -250.8434499350653653 ) ) ;
#63384=CARTESIAN_POINT ( 'NONE',  ( -109.2344962802145147, -291.7711371976793089, -286.1295237892260843 ) ) ;
#63386=CARTESIAN_POINT ( 'NONE',  ( -88.04986210452346995, -292.1236792364506982, -217.5532146111113434 ) ) ;
#63389=CARTESIAN_POINT ( 'NONE',  ( -76.97702002071703475, -292.7390859550529285, -204.7480474552395151 ) ) ;
#63390=CARTESIAN_POINT ( 'NONE',  ( 9.813803242897584767, -278.7174007043979032, -211.5169668397512908 ) ) ;
#63391=CARTESIAN_POINT ( 'NONE',  ( 35.62132981578164959, -293.5215081312270513, -268.0381325303991957 ) ) ;
#63392=CARTESIAN_POINT ( 'NONE',  ( -14.22775861683004273, -280.3437030819081315, -196.8562851808001142 ) ) ;
#63393=CARTESIAN_POINT ( 'NONE',  ( -37.31852028506730079, -282.7185539428414245, -347.3530322087046898 ) ) ;
#63394=CARTESIAN_POINT ( 'NONE',  ( 21.79084572217033156, -286.1823452680244486, -316.2443724027060625 ) ) ;
#63395=CARTESIAN_POINT ( 'NONE',  ( 25.15778577855219567, -280.2378175147488832, -310.5140267591602310 ) ) ;
#63396=CARTESIAN_POINT ( 'NONE',  ( -40.70071967932008761, -284.0098745136969569, -195.3855330098118372 ) ) ;
#63398=CARTESIAN_POINT ( 'NONE',  ( 33.68621961589681746, -279.6736475377336433, -242.3287744070736949 ) ) ;
#63399=CARTESIAN_POINT ( 'NONE',  ( 33.57884248879058475, -286.0985502209837819, -241.0372377868471858 ) ) ;
#63401=CARTESIAN_POINT ( 'NONE',  ( 32.30170494877508247, -295.4754336087215734, -294.9322122211624446 ) ) ;
#63402=CARTESIAN_POINT ( 'NONE',  ( -29.91435360129797516, -275.5696947930615011, -194.3121810011747357 ) ) ;
#63403=CARTESIAN_POINT ( 'NONE',  ( -27.02271926388235102, -276.5840454100101056, -342.6494719591161697 ) ) ;
#63404=CARTESIAN_POINT ( 'NONE',  ( -103.2169436489691208, -291.2403280469488323, -230.3903768987567560 ) ) ;
#63405=CARTESIAN_POINT ( 'NONE',  ( -55.38250664504730025, -281.3623541608585583, -343.7357968260704411 ) ) ;
#63407=CARTESIAN_POINT ( 'NONE',  ( -55.05771012719652191, -290.8774180103706612, -199.3009221124509907 ) ) ;
#63408=CARTESIAN_POINT ( 'NONE',  ( -93.18004292028670932, -293.8543926375297133, -320.4510112440859757 ) ) ;
#63411=CARTESIAN_POINT ( 'NONE',  ( 26.29123287527274044, -292.5675825573036377, -234.3574085703215815 ) ) ;
#63413=CARTESIAN_POINT ( 'NONE',  ( -37.30987171927208834, -271.5523547857346784, -200.3611179825600459 ) ) ;
#63414=CARTESIAN_POINT ( 'NONE',  ( -112.9053835206017595, -295.7805825568702858, -256.8352181784918002 ) ) ;
#63415=CARTESIAN_POINT ( 'NONE',  ( 36.78126115972154508, -279.4915616319282776, -254.6116388800126344 ) ) ;
#63416=CARTESIAN_POINT ( 'NONE',  ( -100.5982566196063033, -286.4395172795497615, -227.2337231558821600 ) ) ;
#63417=CARTESIAN_POINT ( 'NONE',  ( 11.13564330270977365, -286.5788372088599658, -215.7134671445068079 ) ) ;
#63418=CARTESIAN_POINT ( 'NONE',  ( -3.532291924242987324, -278.1174992233793546, -335.8411276878217109 ) ) ;
#63419=CARTESIAN_POINT ( 'NONE',  ( -110.9897807612209277, -294.4154136088573068, -282.5187091491648630 ) ) ;
#63420=CARTESIAN_POINT ( 'NONE',  ( -72.58766957388525043, -297.2856104660420442, -335.4578052676396851 ) ) ;
#63421=CARTESIAN_POINT ( 'NONE',  ( -109.2733383077971041, -277.5393716156920618, -255.7045796643695894 ) ) ;
#63424=CARTESIAN_POINT ( 'NONE',  ( -99.90189105279193882, -296.8134374587357343, -225.5061650450461457 ) ) ;
#63425=CARTESIAN_POINT ( 'NONE',  ( 23.94916730868969523, -290.0495163960730451, -312.6298241657378867 ) ) ;
#63427=CARTESIAN_POINT ( 'NONE',  ( -3.311537114643715807, -289.2420469840506598, -335.1152577459354802 ) ) ;
#63429=CARTESIAN_POINT ( 'NONE',  ( -68.56580941317044164, -278.7105403515757303, -200.2192135571431777 ) ) ;
#63430=CARTESIAN_POINT ( 'NONE',  ( -85.15952346178548282, -298.0627449385340242, -210.1384598056344828 ) ) ;
#63431=CARTESIAN_POINT ( 'NONE',  ( -103.5193828768155129, -289.1777917244504579, -233.4718270675326153 ) ) ;
#63433=CARTESIAN_POINT ( 'NONE',  ( -95.56272344187836154, -296.2049341759523031, -320.7203945448667923 ) ) ;
#63434=CARTESIAN_POINT ( 'NONE',  ( 17.09916428460538285, -294.5815578933360257, -319.0449458822104702 ) ) ;
#63437=CARTESIAN_POINT ( 'NONE',  ( 29.76228481224210043, -289.5477299558951358, -306.8002171729538077 ) ) ;
#63438=CARTESIAN_POINT ( 'NONE',  ( -55.63300648810263738, -276.3376638359844719, -190.3683826091709363 ) ) ;
#63439=CARTESIAN_POINT ( 'NONE',  ( 39.53908953109786495, -280.8595259618310251, -267.0700248326328961 ) ) ;
#63440=CARTESIAN_POINT ( 'NONE',  ( -99.64725244132328896, -287.1135753172270029, -228.9117925661760182 ) ) ;
#63441=CARTESIAN_POINT ( 'NONE',  ( -2.475450634261491256, -285.0789096323716194, -202.3541908783233794 ) ) ;
#63442=CARTESIAN_POINT ( 'NONE',  ( -99.48851566804796676, -289.1904288329418478, -229.2908617249132703 ) ) ;
#63443=CARTESIAN_POINT ( 'NONE',  ( -12.25249928554282342, -278.5897376470998097, -341.9062764110363446 ) ) ;
#63445=CARTESIAN_POINT ( 'NONE',  ( -80.81938008473255763, -277.6611140641101088, -329.0014739295272079 ) ) ;
#63446=CARTESIAN_POINT ( 'NONE',  ( -36.99953479745897766, -279.4051341648615789, -197.2599853547728515 ) ) ;
#63447=CARTESIAN_POINT ( 'NONE',  ( 32.74287989804032861, -277.0308448625507936, -301.5002276593469333 ) ) ;
#63448=CARTESIAN_POINT ( 'NONE',  ( -111.7929223867247401, -277.1197530511220180, -288.4445316558101240 ) ) ;
#63449=CARTESIAN_POINT ( 'NONE',  ( -113.3917889056992436, -270.8501404346486652, -270.3394472961810493 ) ) ;
#63450=CARTESIAN_POINT ( 'NONE',  ( -66.15007414649615214, -274.6254463306890443, -199.1929472639433243 ) ) ;
#63451=CARTESIAN_POINT ( 'NONE',  ( -59.99088444011947274, -299.1896602990232736, -197.3291652706923003 ) ) ;
#63452=CARTESIAN_POINT ( 'NONE',  ( -85.33152481854864391, -293.9090924074130839, -210.2361428286349110 ) ) ;
#63454=CARTESIAN_POINT ( 'NONE',  ( 82.63349580044121012, -300.7641721541951370, -193.1664502239968897 ) ) ;
#63455=CARTESIAN_POINT ( 'NONE',  ( 14.31088586477970281, -289.3845567966654926, -322.3826177067371077 ) ) ;
#63456=CARTESIAN_POINT ( 'NONE',  ( 34.87882036094710969, -289.0091572631905592, -246.5673664989975862 ) ) ;
#63457=CARTESIAN_POINT ( 'NONE',  ( -26.46790819163601327, -288.2588489968362637, -342.7009185497882413 ) ) ;
#63458=CARTESIAN_POINT ( 'NONE',  ( -97.12854247041207145, -283.4095930436573667, -318.8076470488693985 ) ) ;
#63459=CARTESIAN_POINT ( 'NONE',  ( 29.70794543208570460, -279.5391046955959382, -239.4037654485818223 ) ) ;
#63460=CARTESIAN_POINT ( 'NONE',  ( -92.45388373561425510, -287.1136277388338272, -220.5511347061224114 ) ) ;
#63461=CARTESIAN_POINT ( 'NONE',  ( 9.734180712776103306, -279.1933545875294840, -213.5974117790156583 ) ) ;
#63463=CARTESIAN_POINT ( 'NONE',  ( -108.6464988376608289, -279.6333825968851556, -288.2137677879306921 ) ) ;
#63464=CARTESIAN_POINT ( 'NONE',  ( 9.708459146132552675, -276.8761381028799065, -326.2562962516623770 ) ) ;
#63465=CARTESIAN_POINT ( 'NONE',  ( -5.804062505380270132, -287.4415526140517159, -340.1707601035203083 ) ) ;
#63466=CARTESIAN_POINT ( 'NONE',  ( 17.71772245008054725, -283.0920284130585287, -324.0339728135249402 ) ) ;
#63467=CARTESIAN_POINT ( 'NONE',  ( -112.4636465300569910, -284.8364758898206333, -286.9809877877719373 ) ) ;
#63468=CARTESIAN_POINT ( 'NONE',  ( 7.795626209133624585, -282.5828587568330477, -327.7983346106207136 ) ) ;
#63471=PLANE ( 'NONE',  #65591 ) ;
#63472=CARTESIAN_POINT ( 'NONE',  ( -104.9133894839825416, -292.8622579405289343, -235.9762545252293080 ) ) ;
#63473=CARTESIAN_POINT ( 'NONE',  ( -3.524145681270232977, -291.1740041986148526, -201.7196266523338011 ) ) ;
#63474=CARTESIAN_POINT ( 'NONE',  ( 35.93406110213977911, -274.6271962164046840, -271.6008724313213634 ) ) ;
#63475=CARTESIAN_POINT ( 'NONE',  ( 38.71450315925660846, -293.0428461013116248, -281.7086608053122632 ) ) ;
#63477=CARTESIAN_POINT ( 'NONE',  ( -66.62215398130057054, -287.9225393099275152, -338.0422975230064253 ) ) ;
#63478=CARTESIAN_POINT ( 'NONE',  ( 34.29456961880003263, -291.5497233487307653, -251.7541603490146542 ) ) ;
#63479=CARTESIAN_POINT ( 'NONE',  ( -58.79058938073196572, -290.5407935632852627, -340.6073362785776339 ) ) ;
#63481=CARTESIAN_POINT ( 'NONE',  ( -105.8927239133560647, -292.1521867690851195, -300.9150203858601458 ) ) ;
#63482=CARTESIAN_POINT ( 'NONE',  ( -87.40891630622529362, -289.3554763264990584, -214.2959568920143738 ) ) ;
#63483=CARTESIAN_POINT ( 'NONE',  ( -8.935721882019969087, -294.4238225140535405, -200.9348435521304737 ) ) ;
#63484=CARTESIAN_POINT ( 'NONE',  ( -35.94094786127367769, -287.0114029018113229, -197.1392200154339491 ) ) ;
#63485=CARTESIAN_POINT ( 'NONE',  ( 32.74396599752798664, -295.1980916628122600, -243.0507376597385019 ) ) ;
#63488=CARTESIAN_POINT ( 'NONE',  ( 37.74377208733400835, -277.6134522826981765, -276.7312563652594690 ) ) ;
#63489=CARTESIAN_POINT ( 'NONE',  ( -107.6211904154694992, -296.1479739792430905, -239.1659288299988475 ) ) ;
#63490=CARTESIAN_POINT ( 'NONE',  ( 14.21842321400900389, -273.0285999412687374, -217.2618930054013049 ) ) ;
#63491=CARTESIAN_POINT ( 'NONE',  ( -111.7199265676652402, -276.5927671492967193, -273.3932173955231519 ) ) ;
#63492=CARTESIAN_POINT ( 'NONE',  ( -69.67965915161632040, -274.8216527840484673, -204.4719161937341880 ) ) ;
#63493=CARTESIAN_POINT ( 'NONE',  ( -110.8291434654652505, -297.9267994205091554, -274.2303023187665758 ) ) ;
#63495=CARTESIAN_POINT ( 'NONE',  ( -60.57684897720904615, -298.5458866157442230, -200.9336885025287529 ) ) ;
#63498=CARTESIAN_POINT ( 'NONE',  ( 20.83672661848881802, -284.9148030687157416, -222.4687650643165853 ) ) ;
#63499=CARTESIAN_POINT ( 'NONE',  ( -107.9395334423564066, -272.6330337193019204, -251.5945820704199605 ) ) ;
#63500=CARTESIAN_POINT ( 'NONE',  ( -46.50549779701704267, -285.9388967164653081, -193.9083560162137019 ) ) ;
#63501=AXIS2_PLACEMENT_3D ( 'NONE', #50886, #41422, #45148 ) ;
#63502=CARTESIAN_POINT ( 'NONE',  ( 5.542024480287892629, -288.1552058773006593, -334.2886586451904236 ) ) ;
#63503=CARTESIAN_POINT ( 'NONE',  ( -96.95741075061937408, -297.9033412845108728, -316.4520482590865527 ) ) ;
#63504=CARTESIAN_POINT ( 'NONE',  ( 21.11019634088313879, -292.1961249530592681, -317.1084472769126705 ) ) ;
#63506=CARTESIAN_POINT ( 'NONE',  ( 17.11590126150796465, -280.0016126334721775, -216.0783035972525283 ) ) ;
#63507=CARTESIAN_POINT ( 'NONE',  ( -69.85430415644619018, -295.1237833571632905, -202.7746430608542312 ) ) ;
#63509=CARTESIAN_POINT ( 'NONE',  ( -72.56281592650945811, -288.3244551162549101, -334.7552443248590635 ) ) ;
#63510=CARTESIAN_POINT ( 'NONE',  ( 115.2448031289451222, -299.5541904835127980, -192.4725777504219764 ) ) ;
#63511=CARTESIAN_POINT ( 'NONE',  ( 4.715632006333960291, -286.4845634660563860, -332.5218879349656618 ) ) ;
#63512=CARTESIAN_POINT ( 'NONE',  ( -96.85262479312437733, -274.6761594956954013, -226.8118680660714688 ) ) ;
#63513=CARTESIAN_POINT ( 'NONE',  ( -28.31278078357101435, -281.5897110582178584, -194.4324480135501005 ) ) ;
#63514=CARTESIAN_POINT ( 'NONE',  ( -111.9692483712619122, -294.7069538468271048, -259.8211879118365459 ) ) ;
#63515=CARTESIAN_POINT ( 'NONE',  ( -1.252006348918950795, -282.5589870264482215, -333.8160941698243960 ) ) ;
#63516=CARTESIAN_POINT ( 'NONE',  ( -111.9681222818362158, -296.4808446223850069, -289.3852961257915695 ) ) ;
#63517=CARTESIAN_POINT ( 'NONE',  ( -110.4733397539654760, -274.0846547869002165, -262.1673275134239702 ) ) ;
#63518=CARTESIAN_POINT ( 'NONE',  ( 37.14160967504894728, -285.4690400418269860, -257.5745972863552993 ) ) ;
#63519=CARTESIAN_POINT ( 'NONE',  ( 17.67526877177949984, -282.8394078387713080, -219.3892259008433996 ) ) ;
#63520=CARTESIAN_POINT ( 'NONE',  ( -110.4962142403251590, -271.5445183617832754, -264.8766913285733153 ) ) ;
#63523=CARTESIAN_POINT ( 'NONE',  ( -88.02761849207243472, -285.7448040222273562, -325.2294788307875137 ) ) ;
#63525=CARTESIAN_POINT ( 'NONE',  ( -85.33152481854864391, -293.1952119285920162, -330.4860931364850671 ) ) ;
#63526=CARTESIAN_POINT ( 'NONE',  ( -6.648613222671792222, -275.8565030084237719, -340.8174700780544981 ) ) ;
#63527=CARTESIAN_POINT ( 'NONE',  ( 2.242282885843235096, -292.4316107313379121, -208.9652089898891916 ) ) ;
#63528=CARTESIAN_POINT ( 'NONE',  ( -13.28491113351632968, -284.2542170530506382, -340.0713828620420713 ) ) ;
#63529=CARTESIAN_POINT ( 'NONE',  ( 35.90264312936438529, -277.2755653046600059, -279.8087547624083413 ) ) ;
#63530=CARTESIAN_POINT ( 'NONE',  ( -87.91783460465950384, -285.1679985562252000, -327.7088054837951177 ) ) ;
#63531=CARTESIAN_POINT ( 'NONE',  ( -8.351452149322609486, -281.4588251740967735, -337.7903106794484529 ) ) ;
#63532=CARTESIAN_POINT ( 'NONE',  ( -98.03888760067734154, -281.1523823497943795, -226.3060151704531506 ) ) ;
#63533=CARTESIAN_POINT ( 'NONE',  ( 9.508660332924277370, -274.8432997001667104, -209.2542957025698627 ) ) ;
#63534=CARTESIAN_POINT ( 'NONE',  ( 39.62331646840029720, -275.4315580328646433, -274.0460811728977433 ) ) ;
#63536=CARTESIAN_POINT ( 'NONE',  ( -76.39306964733597738, -297.4984922509403873, -333.7955251545253645 ) ) ;
#63539=CARTESIAN_POINT ( 'NONE',  ( -67.75248974617781528, -293.5865982181844061, -339.7548450588759579 ) ) ;
#63540=CARTESIAN_POINT ( 'NONE',  ( 35.44011158421625396, -274.9683292407249269, -263.4211312380294316 ) ) ;
#63541=CARTESIAN_POINT ( 'NONE',  ( 38.91471928111801759, -295.1072153258937760, -273.1299173373506051 ) ) ;
#63542=CARTESIAN_POINT ( 'NONE',  ( 17.28918780799027743, -295.4989021673561638, -324.1345762994708366 ) ) ;
#63543=CARTESIAN_POINT ( 'NONE',  ( -92.11809222832076216, -293.2675844129392431, -219.3561340634631733 ) ) ;
#63544=CARTESIAN_POINT ( 'NONE',  ( -111.7292988090824224, -276.4411255325180719, -278.9762012215477966 ) ) ;
#63545=CARTESIAN_POINT ( 'NONE',  ( -105.7753005641902888, -280.8582068985479623, -241.0668092086709464 ) ) ;
#63546=CARTESIAN_POINT ( 'NONE',  ( -99.95756674138739584, -294.0845780357494164, -310.7118647824431150 ) ) ;
#63547=CARTESIAN_POINT ( 'NONE',  ( -100.3780759615394516, -285.8492128994921018, -312.4875889980253305 ) ) ;
#63548=CARTESIAN_POINT ( 'NONE',  ( -110.6178915127884608, -283.5013314358732259, -268.1643365109780461 ) ) ;
#63549=CARTESIAN_POINT ( 'NONE',  ( 187.0472849604405781, 261.5718128686381760, -152.6093149707159569 ) ) ;
#63550=ORIENTED_EDGE ( 'NONE', *, *, #73502, .F. ) ;
#63551=CARTESIAN_POINT ( 'NONE',  ( -110.3401169112278808, -284.1756953226254154, -273.6348520302908014 ) ) ;
#63553=CARTESIAN_POINT ( 'NONE',  ( 34.03167829427027868, -282.2730222910362272, -242.1567798322602130 ) ) ;
#63554=CARTESIAN_POINT ( 'NONE',  ( -112.6051703620723003, -283.5297988000982059, -255.8229296987388182 ) ) ;
#63555=CARTESIAN_POINT ( 'NONE',  ( -111.1144529447006448, -279.7602976436205040, -249.1384613371601802 ) ) ;
#63557=CARTESIAN_POINT ( 'NONE',  ( -53.96121231241312444, -278.7817454314504175, -344.8900885684331001 ) ) ;
#63558=CARTESIAN_POINT ( 'NONE',  ( -77.44644497616656054, -280.1808219814556082, -204.6875642340633874 ) ) ;
#63560=CARTESIAN_POINT ( 'NONE',  ( -105.5795714935544112, -276.2666405000204009, -254.7536222014695397 ) ) ;
#63561=CARTESIAN_POINT ( 'NONE',  ( -47.24013756723644519, -155.4399423264042071, -365.2501074656324818 ) ) ;
#63563=CARTESIAN_POINT ( 'NONE',  ( 14.75516282931950052, -276.7882957715298176, -216.6401230650349419 ) ) ;
#63564=CARTESIAN_POINT ( 'NONE',  ( -31.81167078611810695, -123.9956632658876146, -363.9854646715294280 ) ) ;
#63566=CARTESIAN_POINT ( 'NONE',  ( -70.44758232897444827, -277.6336853112175049, -203.4451894397258513 ) ) ;
#63567=CARTESIAN_POINT ( 'NONE',  ( 36.80020992900830379, -295.5239366589992187, -287.0617739621884539 ) ) ;
#63568=CARTESIAN_POINT ( 'NONE',  ( 10.35176132541909766, -293.7216967948251636, -325.7617172793203508 ) ) ;
#63569=CARTESIAN_POINT ( 'NONE',  ( -89.45440923371522501, -289.2709095125413796, -326.9631714149327308 ) ) ;
#63571=CARTESIAN_POINT ( 'NONE',  ( 30.37173277726344267, -292.5871970033860521, -305.7658817230463342 ) ) ;
#63572=CARTESIAN_POINT ( 'NONE',  ( -79.75254850530826900, -283.8683700503522118, -209.9017007766233291 ) ) ;
#63573=CARTESIAN_POINT ( 'NONE',  ( -38.94765747131378930, -293.8922084227853588, -196.1432873476060195 ) ) ;
#63574=CARTESIAN_POINT ( 'NONE',  ( 2.841125475369175923, -285.0821094715004165, -208.5869463730107327 ) ) ;
#63575=CARTESIAN_POINT ( 'NONE',  ( -102.6844519964159588, -286.3215390767849726, -236.7223270575540823 ) ) ;
#63577=CARTESIAN_POINT ( 'NONE',  ( -111.0097469576136575, -291.7649438751481625, -248.7778121772562372 ) ) ;
#63578=CARTESIAN_POINT ( 'NONE',  ( 35.20166298559555429, -282.1644260867324761, -279.4596837621922418 ) ) ;
#63579=CARTESIAN_POINT ( 'NONE',  ( -8.551585269441503101, -293.4786751454732325, -341.4041887609004675 ) ) ;
#63580=CARTESIAN_POINT ( 'NONE',  ( -69.28083974303591219, -290.2645762096418025, -340.2614901387378836 ) ) ;
#63581=CARTESIAN_POINT ( 'NONE',  ( -87.33968151546935133, -290.2197185975394405, -328.9095370581140969 ) ) ;
#63582=CARTESIAN_POINT ( 'NONE',  ( 34.01112987939171717, -287.9229723422158145, -285.8396637892997205 ) ) ;
#63585=CARTESIAN_POINT ( 'NONE',  ( -112.3817357046219740, -298.5466424332565225, -259.8124665686835328 ) ) ;
#63586=CARTESIAN_POINT ( 'NONE',  ( -3.663580564556140118, -297.1503186028055552, -193.8616065276860070 ) ) ;
#63588=CARTESIAN_POINT ( 'NONE',  ( 13.50706971362714448, -279.8438260783021860, -217.5854926527914870 ) ) ;
#63589=CARTESIAN_POINT ( 'NONE',  ( -32.68006188642020504, -273.6170480296686947, -193.5508683744300527 ) ) ;
#63590=CARTESIAN_POINT ( 'NONE',  ( -84.94055180905242253, -294.2022650195208371, -326.6869733843120116 ) ) ;
#63591=CARTESIAN_POINT ( 'NONE',  ( 26.13350792768045139, -276.7946931963322186, -232.1978456819760197 ) ) ;
#63592=CARTESIAN_POINT ( 'NONE',  ( -35.76641730591592250, -296.3119934201538967, -196.3482578600380748 ) ) ;
#63593=CARTESIAN_POINT ( 'NONE',  ( -47.83471425619570994, -296.3935046237718893, -343.0558249699116686 ) ) ;
#63594=CARTESIAN_POINT ( 'NONE',  ( -2.986777450175233994, -295.6665421648442020, -335.1219499884488187 ) ) ;
#63596=CARTESIAN_POINT ( 'NONE',  ( -19.45508608312137966, -296.4260678229265977, -344.4864124382992827 ) ) ;
#63597=CARTESIAN_POINT ( 'NONE',  ( -96.83929914791860938, -293.9239326507102987, -316.2965524691065298 ) ) ;
#63598=CARTESIAN_POINT ( 'NONE',  ( -34.86212271287116238, -292.7355360786215215, -197.3012496258579347 ) ) ;
#63599=CARTESIAN_POINT ( 'NONE',  ( -44.03889511919753375, -274.7724858189113775, -193.7618148407555054 ) ) ;
#63600=CARTESIAN_POINT ( 'NONE',  ( -97.23039852896205559, -289.7206124650849688, -227.5114321755981166 ) ) ;
#63601=CARTESIAN_POINT ( 'NONE',  ( -88.72148850990205915, -275.3316383894008368, -215.6537546093924789 ) ) ;
#63602=CARTESIAN_POINT ( 'NONE',  ( -113.4843341027583818, -273.1871977505134055, -258.9600484469769412 ) ) ;
#63603=CARTESIAN_POINT ( 'NONE',  ( -96.42302294119896544, -296.2847928861135642, -313.2949832391473137 ) ) ;
#63604=CARTESIAN_POINT ( 'NONE',  ( -81.30024790682465152, -281.4376555876295924, -209.1561110198740039 ) ) ;
#63605=CARTESIAN_POINT ( 'NONE',  ( 1.140507894786421783, -279.2391311490027874, -204.1765336916885758 ) ) ;
#63606=CARTESIAN_POINT ( 'NONE',  ( -38.55168491383747664, -276.4155416398226635, -347.2496653994394364 ) ) ;
#63607=CARTESIAN_POINT ( 'NONE',  ( 8.086118574069120157, -279.0611655433428950, -209.1174659537655316 ) ) ;
#63608=CARTESIAN_POINT ( 'NONE',  ( 12.44691076144868269, -280.3607973189054974, -326.7431004749354884 ) ) ;
#63609=CARTESIAN_POINT ( 'NONE',  ( -85.68368174464589515, -271.9426698922451351, -214.8096350125262006 ) ) ;
#63610=CARTESIAN_POINT ( 'NONE',  ( -98.97871779457889829, -279.9717813711176859, -313.1798294181111828 ) ) ;
#63613=CARTESIAN_POINT ( 'NONE',  ( 7.270731545534527385, -296.8432417712202778, -194.3875932721223876 ) ) ;
#63614=CARTESIAN_POINT ( 'NONE',  ( 35.49930013023998754, -291.3247551984768506, -251.0085373285693038 ) ) ;
#63615=CARTESIAN_POINT ( 'NONE',  ( -56.18878721987374547, -291.8159877864858345, -195.6483685492484597 ) ) ;
#63616=CARTESIAN_POINT ( 'NONE',  ( -6.024810851595579386, -278.6416711573056659, -338.6932544657472590 ) ) ;
#63617=CARTESIAN_POINT ( 'NONE',  ( 24.72128344378412024, -272.9817730926432091, -228.2288473141829570 ) ) ;
#63619=CARTESIAN_POINT ( 'NONE',  ( -13.84605608623171058, -284.6697458700030552, -342.1752454739954601 ) ) ;
#63621=CARTESIAN_POINT ( 'NONE',  ( -96.25096420031067623, -283.1896048210906542, -223.9220389708277708 ) ) ;
#63623=CARTESIAN_POINT ( 'NONE',  ( -68.70085376097279095, -294.2686422860041375, -336.7355608441679919 ) ) ;
#63624=CARTESIAN_POINT ( 'NONE',  ( 23.75321667938735715, -286.2695566538734511, -312.5531319799890184 ) ) ;
#63626=CARTESIAN_POINT ( 'NONE',  ( -8.484261040513862540, -292.6742987289941311, -339.6011649178135485 ) ) ;
#63627=CARTESIAN_POINT ( 'NONE',  ( -38.73943341945930285, -281.5492694448396946, -346.6549846866687403 ) ) ;
#63628=CARTESIAN_POINT ( 'NONE',  ( -22.04830474426682230, -281.8513427663378366, -198.1106862788269041 ) ) ;
#63629=CARTESIAN_POINT ( 'NONE',  ( -37.99453783505155258, -287.2492129303208799, -193.7609709635084130 ) ) ;
#63630=CARTESIAN_POINT ( 'NONE',  ( 32.62401310169249768, -280.1758766801574438, -300.1395017171752784 ) ) ;
#63631=CARTESIAN_POINT ( 'NONE',  ( 13.13955349035435205, -286.7813699701385417, -217.5595752225050887 ) ) ;
#63632=CARTESIAN_POINT ( 'NONE',  ( -99.66452850903843341, -279.4402355833959177, -309.5873284188227785 ) ) ;
#63633=CARTESIAN_POINT ( 'NONE',  ( -105.4143127907583590, -278.9972528677299692, -297.1700928207763468 ) ) ;
#63634=CARTESIAN_POINT ( 'NONE',  ( -88.78225866803254007, -287.3145523014766241, -215.2240213693260102 ) ) ;
#63637=CARTESIAN_POINT ( 'NONE',  ( -48.96789359179543766, -297.7414090931777650, -194.1902287730759724 ) ) ;
#63639=CARTESIAN_POINT ( 'NONE',  ( -98.68658680091428437, -291.9522714501241012, -312.9118093830333009 ) ) ;
#63641=CARTESIAN_POINT ( 'NONE',  ( 36.57525178469696669, -295.6233781216987495, -234.7283546768995564 ) ) ;
#63643=CARTESIAN_POINT ( 'NONE',  ( 21.34338638418532597, -272.9073228981062584, -223.3716754176242887 ) ) ;
#63644=CARTESIAN_POINT ( 'NONE',  ( -106.4494898238646101, -294.5368695084363821, -302.4633580410126683 ) ) ;
#63645=CARTESIAN_POINT ( 'NONE',  ( -79.75868411222276677, -296.9687054029865863, -210.8734057120314276 ) ) ;
#63646=CARTESIAN_POINT ( 'NONE',  ( 30.06702910626900760, -289.4707491685632590, -300.2664992799170705 ) ) ;
#63647=CARTESIAN_POINT ( 'NONE',  ( 30.94796143133324051, -282.9346893650776451, -241.8217393034181271 ) ) ;
#63648=CARTESIAN_POINT ( 'NONE',  ( -34.66911401790626002, -290.4444504070248172, -346.7251381603615528 ) ) ;
#63649=CARTESIAN_POINT ( 'NONE',  ( -113.6193618540808359, -291.7846663697735607, -276.9280413314039038 ) ) ;
#63650=CARTESIAN_POINT ( 'NONE',  ( -74.56992585627847347, -287.5570800587402118, -205.2381592798225256 ) ) ;
#63651=CARTESIAN_POINT ( 'NONE',  ( -22.56825951563721944, -280.4027918226349811, -194.7373883799859016 ) ) ;
#63652=CARTESIAN_POINT ( 'NONE',  ( 23.70810382217629453, -292.2344658252532668, -314.9052085002197714 ) ) ;
#63653=CARTESIAN_POINT ( 'NONE',  ( 36.47807151846856044, -281.6623156860285917, -292.4452423094710980 ) ) ;
#63654=CARTESIAN_POINT ( 'NONE',  ( 34.09282492035468692, -277.6756924297259843, -290.6060599060998015 ) ) ;
#63655=CARTESIAN_POINT ( 'NONE',  ( -114.2704648735229114, -299.0519495502701943, -270.3937649182068981 ) ) ;
#63656=CARTESIAN_POINT ( 'NONE',  ( -3.200753811961945861, -274.8473952525937420, -338.2605758223133421 ) ) ;
#63658=CARTESIAN_POINT ( 'NONE',  ( 21.85812250357357200, -281.6585488036643028, -313.2003999035796937 ) ) ;
#63659=CARTESIAN_POINT ( 'NONE',  ( -112.0935483623751310, -279.5468013900305095, -287.0993946595646662 ) ) ;
#63660=CARTESIAN_POINT ( 'NONE',  ( -19.16574801169045728, -275.6060272647622469, -199.0982403697296661 ) ) ;
#63661=CARTESIAN_POINT ( 'NONE',  ( -49.29622491187091526, -284.9622309750282625, -194.4793892137579405 ) ) ;
#63662=CARTESIAN_POINT ( 'NONE',  ( -109.6479298844231494, -292.1059518732088236, -286.2244806824243142 ) ) ;
#63663=CARTESIAN_POINT ( 'NONE',  ( -106.1298781139952752, -274.5769215735016360, -237.5796143140116214 ) ) ;
#63664=CARTESIAN_POINT ( 'NONE',  ( -29.90359703394742041, -275.4596142662841771, -194.2166966849506480 ) ) ;
#63666=CARTESIAN_POINT ( 'NONE',  ( 17.43382353512224725, -276.0747326739855225, -318.6359802855083103 ) ) ;
#63667=CARTESIAN_POINT ( 'NONE',  ( -69.27715342387141106, -297.4733591727828639, -338.0520366508173424 ) ) ;
#63668=CARTESIAN_POINT ( 'NONE',  ( -99.05843318894099525, -281.9762871665454895, -312.7725464775796240 ) ) ;
#63669=CARTESIAN_POINT ( 'NONE',  ( -88.63223674173994482, -291.0220872701289068, -212.9588084007271505 ) ) ;
#63670=CARTESIAN_POINT ( 'NONE',  ( 31.79207601991550192, -273.9426320196336064, -298.6475660743995491 ) ) ;
#63671=CARTESIAN_POINT ( 'NONE',  ( -29.04383125834513280, -290.5489164195581111, -346.1609421142818519 ) ) ;
#63672=CARTESIAN_POINT ( 'NONE',  ( -108.6542976877102689, -289.2492470986931039, -287.3534546068873397 ) ) ;
#63674=CARTESIAN_POINT ( 'NONE',  ( -112.5885856976706663, -289.2943231149649819, -257.0753170745582565 ) ) ;
#63675=CARTESIAN_POINT ( 'NONE',  ( -92.43047088025990377, -289.5350012985219905, -318.3669984504579133 ) ) ;
#63677=CARTESIAN_POINT ( 'NONE',  ( 9.610619951405739769, -287.7608868028872848, -209.7230758965140467 ) ) ;
#63678=CARTESIAN_POINT ( 'NONE',  ( -109.1536657757257558, -279.0599576937108282, -257.1274836875249434 ) ) ;
#63679=CARTESIAN_POINT ( 'NONE',  ( -76.93447480514839754, -294.4893377425151471, -336.1032278560408031 ) ) ;
#63680=CARTESIAN_POINT ( 'NONE',  ( -76.69858512047977683, -284.2154580921784941, -336.4860668419599961 ) ) ;
#63682=CARTESIAN_POINT ( 'NONE',  ( -40.81976679879269199, -286.3429391840497829, -193.4086966328136441 ) ) ;
#63683=CARTESIAN_POINT ( 'NONE',  ( 15.84417465479622322, -282.6061953805953522, -320.4675635854309803 ) ) ;
#63684=CARTESIAN_POINT ( 'NONE',  ( -31.07673192236308424, -124.3734504823686962, -364.3838213891494888 ) ) ;
#63685=CARTESIAN_POINT ( 'NONE',  ( 43.83784456572419685, 12.84970072374473737, -330.9960382518970619 ) ) ;
#63686=CARTESIAN_POINT ( 'NONE',  ( -39.93747649349531059, -139.5826026648105085, -361.0100247098301907 ) ) ;
#63687=CARTESIAN_POINT ( 'NONE',  ( -1.634905906460258906, -273.7354602071849854, -206.4904756821619856 ) ) ;
#63688=CARTESIAN_POINT ( 'NONE',  ( 20.10628150010920834, -273.8321851414908110, -224.8003252046226805 ) ) ;
#63689=CARTESIAN_POINT ( 'NONE',  ( 6.573729391164721214, -293.9807122299586126, -333.6000913306708071 ) ) ;
#63690=CARTESIAN_POINT ( 'NONE',  ( -11.55711478694791161, -92.90135622777104629, -356.6579504680683499 ) ) ;
#63691=CARTESIAN_POINT ( 'NONE',  ( 39.13833294582089906, -274.2114841270401939, -268.3355779384526159 ) ) ;
#63692=CARTESIAN_POINT ( 'NONE',  ( -107.8879127575920336, -298.7160927182049477, -247.0874419083096711 ) ) ;
#63693=CARTESIAN_POINT ( 'NONE',  ( -36.21511383969458819, -293.1462426274928248, -197.0481323084369762 ) ) ;
#63695=CARTESIAN_POINT ( 'NONE',  ( -75.67284489018850024, -298.4952808069903654, -203.7903821163441478 ) ) ;
#63696=CARTESIAN_POINT ( 'NONE',  ( 17.87615561098969152, -288.7264212935947967, -318.2801268898141984 ) ) ;
#63697=CARTESIAN_POINT ( 'NONE',  ( -98.14040841507191715, -296.7264721508881280, -317.3470296139737457 ) ) ;
#63698=CARTESIAN_POINT ( 'NONE',  ( -103.0597634418432307, -296.5216504262801891, -310.3694053417344776 ) ) ;
#63699=CARTESIAN_POINT ( 'NONE',  ( 21.80346220801986945, -293.1199825662564535, -227.5514318310680437 ) ) ;
#63701=CARTESIAN_POINT ( 'NONE',  ( 35.19641342558200847, -277.1998366912591223, -249.0234314943387233 ) ) ;
#63704=CARTESIAN_POINT ( 'NONE',  ( 30.67034995205150238, -280.5936670031093172, -234.2768650438665929 ) ) ;
#63705=CARTESIAN_POINT ( 'NONE',  ( -4.008259465461589066, -275.4442166790726105, -205.1374542664041769 ) ) ;
#63706=CARTESIAN_POINT ( 'NONE',  ( 32.76979212578559242, -276.9331675882158379, -240.9276603867034794 ) ) ;
#63707=CARTESIAN_POINT ( 'NONE',  ( -28.81278724125510138, -274.9647697364574697, -345.2845329032169275 ) ) ;
#63708=CARTESIAN_POINT ( 'NONE',  ( -88.20261373559930007, -297.9687287417392554, -217.7827221894572460 ) ) ;
#63709=CARTESIAN_POINT ( 'NONE',  ( -90.84804216980678859, -294.4043526758500775, -320.9562648391395783 ) ) ;
#63711=CARTESIAN_POINT ( 'NONE',  ( -110.6061385808732780, -278.7469560954016288, -294.0240732530908190 ) ) ;
#63712=CARTESIAN_POINT ( 'NONE',  ( 26.76777047168038948, -276.1966812995781879, -305.3806301853728087 ) ) ;
#63713=CARTESIAN_POINT ( 'NONE',  ( 38.48871946633914831, -286.1092089911608696, -260.2099733851670749 ) ) ;
#63714=CARTESIAN_POINT ( 'NONE',  ( -109.1304039746951986, -274.8341690070667482, -248.4720392225015644 ) ) ;
#63716=CARTESIAN_POINT ( 'NONE',  ( 34.72826240167805878, -286.5798283089247320, -257.4845635184381649 ) ) ;
#63717=CARTESIAN_POINT ( 'NONE',  ( -92.03067547374351420, -277.4973931828174045, -220.4903851839320339 ) ) ;
#63718=CARTESIAN_POINT ( 'NONE',  ( -108.5380785521290363, -277.3712424963451895, -251.6984852186540138 ) ) ;
#63719=CARTESIAN_POINT ( 'NONE',  ( -94.54401026523802898, -281.9691851961850944, -317.9973428115391698 ) ) ;
#63720=CARTESIAN_POINT ( 'NONE',  ( -74.39005688471782207, -287.5597041575051094, -205.1359047472036252 ) ) ;
#63721=CARTESIAN_POINT ( 'NONE',  ( -11.09780799893162317, -277.9073718091227079, -338.9059108617805691 ) ) ;
#63723=CARTESIAN_POINT ( 'NONE',  ( -98.41756170676512738, -293.1441825838879822, -226.8325091971890117 ) ) ;
#63724=CARTESIAN_POINT ( 'NONE',  ( -88.54602570495654845, -275.9985925782652885, -326.5046042829356452 ) ) ;
#63725=CARTESIAN_POINT ( 'NONE',  ( -34.04437078377078763, -274.7461334701972078, -197.3335869576112316 ) ) ;
#63726=CARTESIAN_POINT ( 'NONE',  ( 22.80383219056214017, -284.1669401045190853, -315.4448553135704856 ) ) ;
#63728=CARTESIAN_POINT ( 'NONE',  ( 38.13770408471518181, -289.4151841304492905, -265.8789775539829634 ) ) ;
#63729=CARTESIAN_POINT ( 'NONE',  ( -7.258204104566812198, -292.6575793450151650, -339.1179434068606611 ) ) ;
#63731=CARTESIAN_POINT ( 'NONE',  ( -48.93683761338657234, -272.5863141585922449, -197.7369036391480108 ) ) ;
#63732=CARTESIAN_POINT ( 'NONE',  ( 33.81983940537519118, -291.4145406229175705, -249.0437582118194939 ) ) ;
#63733=CARTESIAN_POINT ( 'NONE',  ( -113.2098679957031493, -271.2709011634024137, -296.4525692007673570 ) ) ;
#63735=CARTESIAN_POINT ( 'NONE',  ( -107.7201381255608368, -289.4105309400522970, -240.8724215698831586 ) ) ;
#63736=CARTESIAN_POINT ( 'NONE',  ( 19.54325550619518737, -285.0998133111575612, -219.9040976386709758 ) ) ;
#63737=CARTESIAN_POINT ( 'NONE',  ( -107.9252669706393561, -286.2527566660064622, -249.3675327935352470 ) ) ;
#63738=CARTESIAN_POINT ( 'NONE',  ( -105.7194745871824324, -285.7016360030070814, -244.3403246303864194 ) ) ;
#63739=CARTESIAN_POINT ( 'NONE',  ( -63.83466660808178972, -293.6884461325701068, -199.7616146812952991 ) ) ;
#63740=CARTESIAN_POINT ( 'NONE',  ( 37.70434537338154968, -273.7497022758938670, -279.5966210289873288 ) ) ;
#63741=CARTESIAN_POINT ( 'NONE',  ( 20.80706618780867601, -276.5674423442608827, -320.8237625279735994 ) ) ;
#63742=CARTESIAN_POINT ( 'NONE',  ( -107.4712194354002435, -288.2682441628352308, -298.4887683905960216 ) ) ;
#63743=CARTESIAN_POINT ( 'NONE',  ( 18.90321009041295497, -276.2694000751052386, -322.9492352193798865 ) ) ;
#63744=CARTESIAN_POINT ( 'NONE',  ( -91.58554430201388641, -297.8089678893813925, -321.7137113574090677 ) ) ;
#63747=CARTESIAN_POINT ( 'NONE',  ( -92.04322998459038274, -282.5390839857075775, -319.4614828439005123 ) ) ;
#63748=CARTESIAN_POINT ( 'NONE',  ( -4.509517342370576998, -278.4845707405439725, -202.9151682825841760 ) ) ;
#63750=CARTESIAN_POINT ( 'NONE',  ( 30.64144728577259613, -273.5816689302036480, -235.7056794681675171 ) ) ;
#63751=CARTESIAN_POINT ( 'NONE',  ( -83.07698397872601959, -277.0457044972561107, -327.4541297975299017 ) ) ;
#63752=CARTESIAN_POINT ( 'NONE',  ( 35.89823626676859192, -295.1848101735887440, -278.9725172894914635 ) ) ;
#63753=CARTESIAN_POINT ( 'NONE',  ( 39.33219139450238799, -280.4313367002683322, -267.0843536968103535 ) ) ;
#63754=CARTESIAN_POINT ( 'NONE',  ( -82.49549168579201819, -296.6272288680765428, -328.0846212851636778 ) ) ;
#63755=CARTESIAN_POINT ( 'NONE',  ( -33.44310843291610524, -296.3192385725066629, -346.7816087142763308 ) ) ;
#63756=CARTESIAN_POINT ( 'NONE',  ( -72.84502542494871591, -297.4010674665589136, -206.5762146167980120 ) ) ;
#63757=CARTESIAN_POINT ( 'NONE',  ( -22.36549584848196304, -294.2441040320430830, -196.8715680377788146 ) ) ;
#63758=CARTESIAN_POINT ( 'NONE',  ( -78.52425460745261887, -285.6806199053597197, -205.2996300572852135 ) ) ;
#63759=CARTESIAN_POINT ( 'NONE',  ( -89.29829430854913142, -271.4701366504730800, -215.1458851708738393 ) ) ;
#63760=CARTESIAN_POINT ( 'NONE',  ( 32.71291018312218313, -286.9754881330266585, -238.2741641205226415 ) ) ;
#63761=CARTESIAN_POINT ( 'NONE',  ( -108.8090316680152654, -280.8110248899912449, -248.8142544969474841 ) ) ;
#63763=CARTESIAN_POINT ( 'NONE',  ( -54.80085219291658660, -284.8810501478265564, -199.1849130997260602 ) ) ;
#63764=CARTESIAN_POINT ( 'NONE',  ( -92.14914908545156891, -287.8345793509295731, -321.6331060379923201 ) ) ;
#63765=CARTESIAN_POINT ( 'NONE',  ( 207.9739649226136180, 291.4638663531892462, -68.48153742335392735 ) ) ;
#63766=CARTESIAN_POINT ( 'NONE',  ( 34.05747892948230060, -286.8555494794040328, -254.8644837746137455 ) ) ;
#63768=CARTESIAN_POINT ( 'NONE',  ( -50.04273765835110765, -284.1515421170400941, -346.1215237110538965 ) ) ;
#63769=CARTESIAN_POINT ( 'NONE',  ( -94.52799409573900391, -290.3077173873032848, -219.1502988574988535 ) ) ;
#63770=CARTESIAN_POINT ( 'NONE',  ( -113.2489331221395048, -280.2439095637512310, -263.1105287173102738 ) ) ;
#63771=CARTESIAN_POINT ( 'NONE',  ( -101.4869556204810408, -280.4195366246457297, -228.5676890210993406 ) ) ;
#63772=CARTESIAN_POINT ( 'NONE',  ( 34.33464662420605862, -281.2020511916978194, -256.4568544086280326 ) ) ;
#63773=CARTESIAN_POINT ( 'NONE',  ( 12.86702739149617436, -276.7526178099279264, -214.5769015516253262 ) ) ;
#63774=CARTESIAN_POINT ( 'NONE',  ( -69.52792029245891570, -295.4641715322786695, -340.3258708293686823 ) ) ;
#63775=CARTESIAN_POINT ( 'NONE',  ( -108.5636036013131900, -288.8623837752676877, -247.9733699220326173 ) ) ;
#63776=CARTESIAN_POINT ( 'NONE',  ( -108.7751547041566056, -295.6889208430971507, -253.8842359332637670 ) ) ;
#63779=CARTESIAN_POINT ( 'NONE',  ( 34.35280635332465238, -283.7319234407000295, -290.3913935670002502 ) ) ;
#63780=CARTESIAN_POINT ( 'NONE',  ( -106.8907132148062971, -295.9219512209721188, -292.7739342437091636 ) ) ;
#63781=CARTESIAN_POINT ( 'NONE',  ( 39.34638038248613867, -294.5950747074009541, -267.4346271081413420 ) ) ;
#63782=CARTESIAN_POINT ( 'NONE',  ( -3.566921220749860844, -283.2454588910824782, -335.2069023307449811 ) ) ;
#63783=CARTESIAN_POINT ( 'NONE',  ( 19.86855022352509081, -273.9139232226220884, -219.0989316371287998 ) ) ;
#63784=CARTESIAN_POINT ( 'NONE',  ( -4.369239354835378286, -289.2803436228336409, -339.8459298248872074 ) ) ;
#63785=CARTESIAN_POINT ( 'NONE',  ( -5.988645452508174927, -280.7840180005426305, -339.3342391686034034 ) ) ;
#63786=CARTESIAN_POINT ( 'NONE',  ( -113.7920368271609988, -290.7672799340705296, -279.8058919025192495 ) ) ;
#63787=CARTESIAN_POINT ( 'NONE',  ( -3.352748113942630059, -288.9239665833383128, -335.0455866819347648 ) ) ;
#63790=CARTESIAN_POINT ( 'NONE',  ( 202.4138562182569672, 292.0436489450776207, -53.99999999998431832 ) ) ;
#63791=CARTESIAN_POINT ( 'NONE',  ( -8.284807207348070079, -284.1987788159655679, -340.9749666555922545 ) ) ;
#63792=CARTESIAN_POINT ( 'NONE',  ( 35.77081079830085031, -291.2666405000204577, -287.0812184334320705 ) ) ;
#63794=CARTESIAN_POINT ( 'NONE',  ( -91.51601861600957477, -278.1777531467093354, -220.9711464265127461 ) ) ;
#63795=CARTESIAN_POINT ( 'NONE',  ( -18.55102464135140039, -273.9543749488533422, -195.6558859789888061 ) ) ;
#63796=CARTESIAN_POINT ( 'NONE',  ( -46.09795327289893407, -279.1634940189329086, -344.7323015913306108 ) ) ;
#63797=CARTESIAN_POINT ( 'NONE',  ( 162.6064035890194646, 217.7902839693395549, -203.4103096416544929 ) ) ;
#63798=CARTESIAN_POINT ( 'NONE',  ( 38.68987013377453366, -280.2291292074517060, -278.4741444403497894 ) ) ;
#63799=CARTESIAN_POINT ( 'NONE',  ( -0.4607812854550503712, -280.5794144521117914, -335.2583030436366016 ) ) ;
#63800=CARTESIAN_POINT ( 'NONE',  ( -109.3778401604835295, -298.0037104908390120, -294.5431059548459416 ) ) ;
#63801=CARTESIAN_POINT ( 'NONE',  ( 18.02316104008952635, -294.7230418898782318, -318.0532549517193388 ) ) ;
#63803=CARTESIAN_POINT ( 'NONE',  ( -57.77610454242650206, -290.4676348550997318, -199.7127135470596500 ) ) ;
#63804=CARTESIAN_POINT ( 'NONE',  ( 21.76717817412899336, -275.5410885884037953, -221.1731794928912223 ) ) ;
#63805=CARTESIAN_POINT ( 'NONE',  ( -90.19660543137686659, -273.2784594614061007, -219.9904813671150521 ) ) ;
#63810=CARTESIAN_POINT ( 'NONE',  ( -62.42759092147420574, -280.7977816206793023, -201.4241203814754329 ) ) ;
#63811=CARTESIAN_POINT ( 'NONE',  ( 21.17581120810025652, -282.6519351503295070, -221.8876728420265749 ) ) ;
#63812=CARTESIAN_POINT ( 'NONE',  ( -109.6515444122650251, -283.7645479020408743, -258.6759517145612222 ) ) ;
#63813=CARTESIAN_POINT ( 'NONE',  ( -6.273742743945875944, -282.3250987886999610, -202.9258257372329979 ) ) ;
#63814=CARTESIAN_POINT ( 'NONE',  ( 36.29368926362795378, -274.0844018883019544, -274.3694596340391172 ) ) ;
#63817=CARTESIAN_POINT ( 'NONE',  ( -75.24762348572066628, -278.3469872631963540, -337.1989799694664498 ) ) ;
#63821=CARTESIAN_POINT ( 'NONE',  ( -44.24291873220152382, -285.1187785616862129, -345.4518581966116244 ) ) ;
#63822=CARTESIAN_POINT ( 'NONE',  ( 22.72634353672973617, -292.1682229093307228, -228.5726439016649465 ) ) ;
#63824=CARTESIAN_POINT ( 'NONE',  ( 38.00674755905752988, -287.0930927040805614, -285.7209427902196239 ) ) ;
#63825=CARTESIAN_POINT ( 'NONE',  ( -109.6501525313736067, -282.9982799642866098, -254.5076713940242996 ) ) ;
#63826=CARTESIAN_POINT ( 'NONE',  ( -79.63319640983496583, -284.0431979902666626, -210.0756156493136757 ) ) ;
#63827=CARTESIAN_POINT ( 'NONE',  ( 23.57130789212449429, -286.3698151807546992, -312.4260393832969953 ) ) ;
#63828=CARTESIAN_POINT ( 'NONE',  ( 35.91523753047317058, -282.6977550788365079, -265.8277319654869757 ) ) ;
#63829=CARTESIAN_POINT ( 'NONE',  ( -5.928139016700665564, -272.4649302086914986, -202.2568682551758172 ) ) ;
#63831=CARTESIAN_POINT ( 'NONE',  ( -110.1554670494622457, -283.2391298779421618, -247.7204685870175638 ) ) ;
#63832=CARTESIAN_POINT ( 'NONE',  ( -102.1351669354357341, -299.0580786989693252, -232.4856098810211904 ) ) ;
#63833=CARTESIAN_POINT ( 'NONE',  ( -111.1920370516100149, -282.7348430719764565, -256.0852206937172468 ) ) ;
#63835=CARTESIAN_POINT ( 'NONE',  ( -16.86738248179304023, -281.2644266761291192, -200.0460359272181279 ) ) ;
#63836=CARTESIAN_POINT ( 'NONE',  ( 37.86847630212764670, -289.5668755342401255, -271.4975313261301721 ) ) ;
#63839=CARTESIAN_POINT ( 'NONE',  ( 37.42333510476321123, -295.3285179475146265, -259.0790458297708483 ) ) ;
#63841=CARTESIAN_POINT ( 'NONE',  ( -99.31543678382014662, -275.9800244515741952, -312.6015797959382780 ) ) ;
#63842=CARTESIAN_POINT ( 'NONE',  ( -91.49200464830124702, -288.9962009914140708, -324.9511423292060499 ) ) ;
#63843=CARTESIAN_POINT ( 'NONE',  ( -15.37391446412879326, -293.1629958653196582, -340.8695105723052734 ) ) ;
#63844=CARTESIAN_POINT ( 'NONE',  ( -30.19788987629874200, -278.8290988925231773, -197.1652965699153128 ) ) ;
#63845=CARTESIAN_POINT ( 'NONE',  ( -104.4937802609203175, -271.0580530685751341, -238.2377257472312522 ) ) ;
#63846=CARTESIAN_POINT ( 'NONE',  ( -4.628515023603078760, -293.8075450568010183, -204.5360756298416050 ) ) ;
#63847=CARTESIAN_POINT ( 'NONE',  ( -110.4683760289727132, -287.2662352645559167, -253.7030783399848985 ) ) ;
#63848=CARTESIAN_POINT ( 'NONE',  ( -111.9187178457651441, -295.2366300057087187, -254.1454466737765188 ) ) ;
#63849=CARTESIAN_POINT ( 'NONE',  ( 1.752452504987862536, -290.1198481316873767, -332.9557475003668401 ) ) ;
#63850=CARTESIAN_POINT ( 'NONE',  ( -44.77530831762304331, -290.1992870000940457, -194.6867032898723266 ) ) ;
#63851=CARTESIAN_POINT ( 'NONE',  ( -110.8943557418349570, -291.9303931852601295, -273.9556923212676907 ) ) ;
#63853=CARTESIAN_POINT ( 'NONE',  ( -107.5531388676546811, -291.6270004388076131, -249.7507281951459674 ) ) ;
#63855=CARTESIAN_POINT ( 'NONE',  ( -96.97126178976934341, -291.1090196875140350, -318.4684305686678840 ) ) ;
#63856=CARTESIAN_POINT ( 'NONE',  ( 37.63876384571953082, -279.6745986813138529, -278.3693361883300099 ) ) ;
#63857=CARTESIAN_POINT ( 'NONE',  ( 24.84787079955360412, -293.0240290120265740, -232.0361438693508092 ) ) ;
#63858=CARTESIAN_POINT ( 'NONE',  ( -45.27337108283251865, -279.9544503059973977, -193.7177326970513036 ) ) ;
#63859=CARTESIAN_POINT ( 'NONE',  ( 17.80816477315422119, -281.9560978229920352, -324.1423692431051222 ) ) ;
#63860=CARTESIAN_POINT ( 'NONE',  ( 6.908704449835291861, -286.4486423060803304, -330.7740870580619799 ) ) ;
#63861=CARTESIAN_POINT ( 'NONE',  ( 21.98296813773478320, -280.3082111784922290, -315.0077722923272745 ) ) ;
#63862=CARTESIAN_POINT ( 'NONE',  ( -57.20117490572079788, -283.7958924556551779, -197.9843088319997548 ) ) ;
#63863=CARTESIAN_POINT ( 'NONE',  ( -5.218093358983717955, -278.9471862940930578, -201.1456454107276670 ) ) ;
#63864=CARTESIAN_POINT ( 'NONE',  ( -2.351619894606735262, -285.4244546327939815, -202.1028391750618880 ) ) ;
#63865=CARTESIAN_POINT ( 'NONE',  ( 3.010500028292293351, -275.4117782673250190, -209.2735199486696729 ) ) ;
#63867=CARTESIAN_POINT ( 'NONE',  ( 33.89420135918904009, -295.4048268992617636, -289.6935827811574882 ) ) ;
#63868=CARTESIAN_POINT ( 'NONE',  ( 38.15646561286266802, -277.1300008898330134, -282.4679599193767672 ) ) ;
#63869=CARTESIAN_POINT ( 'NONE',  ( -89.10380335433531229, -277.4713381324768307, -321.9379933816849757 ) ) ;
#63870=CARTESIAN_POINT ( 'NONE',  ( -73.43559284086877881, -291.7535333634036760, -202.3298162416406569 ) ) ;
#63871=CARTESIAN_POINT ( 'NONE',  ( -49.87911212311918518, -281.2905966865749292, -344.9265872018413006 ) ) ;
#63872=CARTESIAN_POINT ( 'NONE',  ( -62.87155754369371152, -290.7701714296186992, -201.7197687210510537 ) ) ;
#63873=CARTESIAN_POINT ( 'NONE',  ( 30.41203594710298574, -291.9765684371523093, -302.6446823547061626 ) ) ;
#63876=CARTESIAN_POINT ( 'NONE',  ( -60.27233686336654728, -291.2544695448601146, -200.9381976835420005 ) ) ;
#63878=CARTESIAN_POINT ( 'NONE',  ( -105.5795714935544112, -298.8376638359844719, -285.9686137636504668 ) ) ;
#63879=CARTESIAN_POINT ( 'NONE',  ( -113.1552694616390227, -295.7630695077583027, -258.2312289835654724 ) ) ;
#63881=ADVANCED_FACE ( 'NONE', ( #78237 ), #12570, .T. ) ;
#63882=CARTESIAN_POINT ( 'NONE',  ( -95.88209119270837277, -285.1995417971489815, -319.6390812674281392 ) ) ;
#63883=CARTESIAN_POINT ( 'NONE',  ( 24.95182763898558775, -286.8610996736716174, -232.3017380240255818 ) ) ;
#63884=CARTESIAN_POINT ( 'NONE',  ( 35.05100779430772207, -276.8921519726080192, -256.5769388807461837 ) ) ;
#63885=CARTESIAN_POINT ( 'NONE',  ( -109.7647924879880890, -294.8061539525104990, -252.2328422257478167 ) ) ;
#63886=CARTESIAN_POINT ( 'NONE',  ( -107.8275230432567469, -298.0150359777803715, -293.1039117068961559 ) ) ;
#63887=CARTESIAN_POINT ( 'NONE',  ( -21.58264370543693289, -275.6406449344836460, -342.0986934635167813 ) ) ;
#63890=CARTESIAN_POINT ( 'NONE',  ( -105.2329583771384449, -296.6891710807491904, -233.9641532944656888 ) ) ;
#63891=CARTESIAN_POINT ( 'NONE',  ( -23.49377399475570982, -290.7940722046583915, -343.5544519936491952 ) ) ;
#63893=CARTESIAN_POINT ( 'NONE',  ( -13.24646216962237943, -289.3821390969849858, -339.3778708459862514 ) ) ;
#63895=CARTESIAN_POINT ( 'NONE',  ( 6.061120384202320466, -279.6842153298699714, -207.0443320249913768 ) ) ;
#63896=CARTESIAN_POINT ( 'NONE',  ( -87.40220084427529912, -298.0268834631633013, -211.9191841063840798 ) ) ;
#63897=CARTESIAN_POINT ( 'NONE',  ( -110.3580236809855393, -288.4342662246273221, -290.5829373117604177 ) ) ;
#63898=CARTESIAN_POINT ( 'NONE',  ( -111.9471045184252773, -296.6474188180910687, -289.3821338599424848 ) ) ;
#63900=CARTESIAN_POINT ( 'NONE',  ( 35.55548941238512839, -293.8188307166893765, -265.3106526661845237 ) ) ;
#63902=CIRCLE ( 'NONE', #30602, 1.000000000000000888 ) ;
#63905=CARTESIAN_POINT ( 'NONE',  ( 35.29376715004156040, -289.3689962735458039, -293.7448013053996760 ) ) ;
#63906=CARTESIAN_POINT ( 'NONE',  ( -19.05039376806008633, -279.3376638359844719, -350.3538533559490702 ) ) ;
#63908=CARTESIAN_POINT ( 'NONE',  ( 38.69521478830813521, -280.7526989510703288, -258.5394398989590172 ) ) ;
#63909=CARTESIAN_POINT ( 'NONE',  ( -12.90727045389426841, -284.7341782109277233, -341.1478725720385228 ) ) ;
#63910=CARTESIAN_POINT ( 'NONE',  ( 9.464244038540272186, -285.2563462623699024, -209.9640163802309871 ) ) ;
#63911=AXIS2_PLACEMENT_3D ( 'NONE', #52615, #45984, #81497 ) ;
#63912=CARTESIAN_POINT ( 'NONE',  ( -107.0506840028030950, -288.9753708477634859, -244.1003949682119014 ) ) ;
#63913=CARTESIAN_POINT ( 'NONE',  ( -25.93221553894920106, -278.7687428519294031, -345.2619133044655655 ) ) ;
#63914=CARTESIAN_POINT ( 'NONE',  ( -104.4420681256212760, -278.9383619206318485, -241.6114986008234666 ) ) ;
#63915=CARTESIAN_POINT ( 'NONE',  ( 32.07601627227643348, -280.5950732792880444, -247.2870407276015783 ) ) ;
#63916=CARTESIAN_POINT ( 'NONE',  ( 19.65671261876532583, -277.3312506461663247, -321.6903594015559520 ) ) ;
#63917=CARTESIAN_POINT ( 'NONE',  ( -84.31129892726592345, -278.2174077550121751, -209.7806518728222613 ) ) ;
#63918=CARTESIAN_POINT ( 'NONE',  ( -90.76730617333356577, -228.9098355046940867, -345.5290054426631059 ) ) ;
#63919=CARTESIAN_POINT ( 'NONE',  ( -52.51089187581975182, -274.8038067254300358, -195.0558227561601257 ) ) ;
#63920=CARTESIAN_POINT ( 'NONE',  ( -67.95816730762523150, -299.0834443002640342, -200.2959036786763534 ) ) ;
#63921=CARTESIAN_POINT ( 'NONE',  ( -114.2704648735229114, -293.0519495502703080, -270.3937649182068981 ) ) ;
#63923=CARTESIAN_POINT ( 'NONE',  ( 35.93962257626139944, -288.6764844544147763, -273.7605098693581454 ) ) ;
#63924=CARTESIAN_POINT ( 'NONE',  ( -111.3775496909184568, -286.5290943280365923, -253.2536050915478825 ) ) ;
#63925=CARTESIAN_POINT ( 'NONE',  ( 32.37330116776406186, -286.6091009658677535, -248.3257585204912345 ) ) ;
#63926=CARTESIAN_POINT ( 'NONE',  ( -112.9365813393347082, -284.2424117108164410, -255.7682841167352876 ) ) ;
#63927=CARTESIAN_POINT ( 'NONE',  ( 31.82716349144546086, -279.6108167209565636, -244.4829234508656270 ) ) ;
#63928=CARTESIAN_POINT ( 'NONE',  ( -22.23117688646444279, -288.1080109496847399, -197.6272956720659408 ) ) ;
#63929=CARTESIAN_POINT ( 'NONE',  ( -5.239131764100291910, -278.9624145647896967, -204.0276207189525906 ) ) ;
#63930=CARTESIAN_POINT ( 'NONE',  ( -39.15324416686435427, -278.3905360031849341, -343.8319406777193876 ) ) ;
#63931=CARTESIAN_POINT ( 'NONE',  ( 9.519751953192566063, -275.2090770793129764, -214.2413899064675036 ) ) ;
#63932=CARTESIAN_POINT ( 'NONE',  ( 5.323378345878090556, -287.2835517467686373, -333.9826536177548064 ) ) ;
#63933=CARTESIAN_POINT ( 'NONE',  ( -21.74874811472405156, -283.6600031040663907, -345.6008592600969678 ) ) ;
#63934=CARTESIAN_POINT ( 'NONE',  ( -79.12104613906727479, -284.0920160009975461, -334.9677209734464896 ) ) ;
#63935=CARTESIAN_POINT ( 'NONE',  ( 13.92619242967292870, -282.4752263544112338, -322.3996205455611062 ) ) ;
#63939=CARTESIAN_POINT ( 'NONE',  ( -6.113612522359519019, -290.5065484773019762, -339.3909088555104177 ) ) ;
#63940=CARTESIAN_POINT ( 'NONE',  ( -86.18524014526099108, -290.0761294878942635, -211.4059533497838572 ) ) ;
#63941=CARTESIAN_POINT ( 'NONE',  ( -92.18644043809439381, -272.3021030421900264, -221.8280065137352892 ) ) ;
#63942=CARTESIAN_POINT ( 'NONE',  ( 39.12569766671325766, -292.7928488575410597, -261.7455906419088478 ) ) ;
#63943=CARTESIAN_POINT ( 'NONE',  ( -18.31296690027854979, -287.2824853615557572, -341.6084061846958662 ) ) ;
#63944=CARTESIAN_POINT ( 'NONE',  ( 32.48875889757632507, -292.1157054966603823, -295.0436267988609984 ) ) ;
#63945=CARTESIAN_POINT ( 'NONE',  ( 1.534839239654746335, -289.7248591643124769, -332.6166012055394958 ) ) ;
#63946=CARTESIAN_POINT ( 'NONE',  ( -37.37352853689063892, -288.5519495502701943, -195.3611179825600175 ) ) ;
#63947=CARTESIAN_POINT ( 'NONE',  ( -102.0594008324897430, -292.0446285133974698, -308.3665507390087441 ) ) ;
#63948=CARTESIAN_POINT ( 'NONE',  ( -111.1204602315069110, -288.7370523743019248, -255.9163171806554828 ) ) ;
#63949=CARTESIAN_POINT ( 'NONE',  ( -64.34574406780967593, -293.7000612935581785, -200.3370762585978184 ) ) ;
#63950=CARTESIAN_POINT ( 'NONE',  ( -71.29792806797661342, -286.5334382806494773, -205.4736536093269024 ) ) ;
#63951=CARTESIAN_POINT ( 'NONE',  ( 18.98750762650380608, -294.8616755098453268, -220.5717214058626041 ) ) ;
#63952=CARTESIAN_POINT ( 'NONE',  ( -112.5397100641337147, -270.5523142621870534, -270.3356552556126076 ) ) ;
#63954=CARTESIAN_POINT ( 'NONE',  ( -36.97363918710599506, -276.0366581621883597, -194.9940397895167621 ) ) ;
#63955=CARTESIAN_POINT ( 'NONE',  ( -59.56439087084695672, -281.3396374717880235, -342.0477862637842463 ) ) ;
#63956=CARTESIAN_POINT ( 'NONE',  ( -113.7836169506870050, -295.6516053025841870, -278.1580515267068563 ) ) ;
#63957=CARTESIAN_POINT ( 'NONE',  ( -8.556310642217372475, -272.6738577108719710, -202.1201210344045478 ) ) ;
#63958=CARTESIAN_POINT ( 'NONE',  ( -104.4393792924921485, -276.2029107980352478, -302.7173383343444470 ) ) ;
#63959=CARTESIAN_POINT ( 'NONE',  ( -79.09348697847681819, -274.6804055336842794, -209.9344927259447218 ) ) ;
#63960=CARTESIAN_POINT ( 'NONE',  ( 6.908656765525013732, -273.2157517946503162, -208.0024159844666372 ) ) ;
#63961=CARTESIAN_POINT ( 'NONE',  ( -108.5350469604711350, -297.7329041329210781, -289.0356676466272461 ) ) ;
#63963=CARTESIAN_POINT ( 'NONE',  ( -82.05085867560535462, -298.2278221456635947, -212.3858269163354748 ) ) ;
#63965=CARTESIAN_POINT ( 'NONE',  ( 33.51701669605155587, -285.9049048152741079, -296.1535586554102792 ) ) ;
#63966=CARTESIAN_POINT ( 'NONE',  ( -107.1959075243145918, -272.6682334736833013, -248.9891644333909824 ) ) ;
#63968=CARTESIAN_POINT ( 'NONE',  ( -63.20143416468979325, -285.7244031416678354, -197.8333704954370091 ) ) ;
#63969=CARTESIAN_POINT ( 'NONE',  ( 16.28750053660273878, -286.4555227192495295, -215.1374534216471091 ) ) ;
#63970=CARTESIAN_POINT ( 'NONE',  ( -100.9419878495283029, -299.0733041075435494, -229.9456481275238389 ) ) ;
#63971=CARTESIAN_POINT ( 'NONE',  ( -48.08069442457507847, -293.1887845623392650, -344.4724648055770899 ) ) ;
#63974=CARTESIAN_POINT ( 'NONE',  ( -28.23397479790325804, -279.3619652105966225, -194.0107625888133782 ) ) ;
#63975=CARTESIAN_POINT ( 'NONE',  ( -37.37352853689063181, -286.5523547857347353, -345.3611179825600175 ) ) ;
#63978=CARTESIAN_POINT ( 'NONE',  ( -39.98770596539654321, -287.8809283587211780, -343.7603309726471821 ) ) ;
#63980=CARTESIAN_POINT ( 'NONE',  ( -107.9231239757965568, -288.2232244667166015, -295.7237529994458214 ) ) ;
#63981=CARTESIAN_POINT ( 'NONE',  ( -111.0357539742292801, -274.1079617381141134, -267.6306981556637652 ) ) ;
#63982=CARTESIAN_POINT ( 'NONE',  ( -50.85340104127683247, -281.3080300680329060, -195.1544678121706511 ) ) ;
#63983=CARTESIAN_POINT ( 'NONE',  ( -94.35395794113870238, -293.8921346682355988, -319.6359519670539271 ) ) ;
#63984=CARTESIAN_POINT ( 'NONE',  ( -21.38821466200059263, -282.8419486104713769, -341.6485595088821583 ) ) ;
#63985=CARTESIAN_POINT ( 'NONE',  ( -109.8515755478251776, -297.0458897517643777, -244.4513134462553694 ) ) ;
#63986=CARTESIAN_POINT ( 'NONE',  ( -77.90965545200457143, -299.0167050613230799, -208.7778506104841085 ) ) ;
#63987=CARTESIAN_POINT ( 'NONE',  ( 7.334211319854624378, -282.6608750085383122, -210.0548661866774864 ) ) ;
#63988=CARTESIAN_POINT ( 'NONE',  ( -96.60585650401269220, -295.0104656711245639, -313.4077316617878068 ) ) ;
#63989=DIRECTION ( 'NONE',  ( -0.000000000000000000, 0.000000000000000000, 1.000000000000000000 ) ) ;
#63990=CARTESIAN_POINT ( 'NONE',  ( -37.51968410788270347, -285.0343163989131767, -345.0184190254362306 ) ) ;
#63992=CARTESIAN_POINT ( 'NONE',  ( -20.25526795762938548, -286.3380690714490697, -345.3683826091709648 ) ) ;
#63993=CARTESIAN_POINT ( 'NONE',  ( 38.97595581957405386, -274.8668436350243383, -279.7383590416616812 ) ) ;
#63996=CARTESIAN_POINT ( 'NONE',  ( 19.34713351667051384, -292.7345472496355683, -224.3481285050190195 ) ) ;
#63997=CARTESIAN_POINT ( 'NONE',  ( 22.66693542582543586, -282.4803380483452315, -227.5864594530907254 ) ) ;
#63998=CARTESIAN_POINT ( 'NONE',  ( 23.13297719271521302, -277.7367969593358907, -312.7484570792333329 ) ) ;
#64000=CARTESIAN_POINT ( 'NONE',  ( -103.8948131869147034, -285.4852951630426787, -308.0087442827289124 ) ) ;
#64001=CARTESIAN_POINT ( 'NONE',  ( 12.17331818995174331, -281.1395012102180999, -324.5403895253638211 ) ) ;
#64002=CARTESIAN_POINT ( 'NONE',  ( -84.72036587700959842, -281.3998237883651541, -212.1538534874497941 ) ) ;
#64003=CARTESIAN_POINT ( 'NONE',  ( -36.54062426294925103, -298.0619223292007973, -193.3611179782305101 ) ) ;
#64004=CARTESIAN_POINT ( 'NONE',  ( 12.70300882681554810, -276.2095954623048328, -328.8805772256615114 ) ) ;
#64005=CARTESIAN_POINT ( 'NONE',  ( 23.75612834044204291, -294.8907699401158879, -227.8137400918135427 ) ) ;
#64006=DIRECTION ( 'NONE',  ( -1.000000000000000000, -0.000000000000000000, -0.000000000000000000 ) ) ;
#64008=CARTESIAN_POINT ( 'NONE',  ( -108.6797376087111786, -295.0191204664316729, -244.8426954685156147 ) ) ;
#64009=CARTESIAN_POINT ( 'NONE',  ( 22.51264878595645413, -275.6446592090524632, -312.3460000388446360 ) ) ;
#64010=CARTESIAN_POINT ( 'NONE',  ( 22.63880648962044262, -295.7089856591564967, -317.5524876303701376 ) ) ;
#64011=CARTESIAN_POINT ( 'NONE',  ( 37.37060531289780840, -294.5439271686976781, -253.3884559164038990 ) ) ;
#64012=CARTESIAN_POINT ( 'NONE',  ( 31.11216437304329929, -289.9507104260557639, -300.7238162934110619 ) ) ;
#64013=CARTESIAN_POINT ( 'NONE',  ( -57.10836075811388213, -275.3074325443680550, -342.5904730229486859 ) ) ;
#64014=CARTESIAN_POINT ( 'NONE',  ( -24.04890530807592697, -278.8013690487071585, -343.6571236880507172 ) ) ;
#64015=CARTESIAN_POINT ( 'NONE',  ( -58.84716550517746469, -293.4123591213312920, -341.6270225551393196 ) ) ;
#64016=CARTESIAN_POINT ( 'NONE',  ( 25.24663991732245094, -282.8391641673076720, -227.5729509991774080 ) ) ;
#64017=CARTESIAN_POINT ( 'NONE',  ( -83.83333562459020527, -284.3169095373505684, -213.6140109585516882 ) ) ;
#64018=CARTESIAN_POINT ( 'NONE',  ( 155.5793399543505586, 205.2758529659251394, -216.3944369107308034 ) ) ;
#64020=CARTESIAN_POINT ( 'NONE',  ( -110.1171876763455657, -284.1399445133095014, -276.3457565537390224 ) ) ;
#64022=CARTESIAN_POINT ( 'NONE',  ( 26.47233443660443086, -283.1939359025325871, -312.8965326654148953 ) ) ;
#64024=CARTESIAN_POINT ( 'NONE',  ( -111.1132387943987396, -283.0871840292786032, -290.9952838733511271 ) ) ;
#64025=CARTESIAN_POINT ( 'NONE',  ( -74.90329787781249138, -280.5057736683519352, -203.4137760814069225 ) ) ;
#64026=CARTESIAN_POINT ( 'NONE',  ( -94.67693004519308886, -279.3846409035803049, -320.7136667173180058 ) ) ;
#64027=CARTESIAN_POINT ( 'NONE',  ( 34.45848030099739390, -273.0523547857346784, -270.3937649182068412 ) ) ;
#64028=CARTESIAN_POINT ( 'NONE',  ( 200.7966458510228449, 288.9840134172227408, -97.53539858349294889 ) ) ;
#64030=CARTESIAN_POINT ( 'NONE',  ( 12.75541053804829161, -276.7526178115898006, -214.7008287420459567 ) ) ;
#64031=CARTESIAN_POINT ( 'NONE',  ( -104.5909623734931273, -255.9058999860332335, -326.6256074632783566 ) ) ;
#64032=CARTESIAN_POINT ( 'NONE',  ( -62.84780177995892814, -277.7387112948403001, -200.1546915667861981 ) ) ;
#64033=CARTESIAN_POINT ( 'NONE',  ( -40.61154822904870088, -293.7717267207963801, -194.4318258477070174 ) ) ;
#64034=CARTESIAN_POINT ( 'NONE',  ( 18.90622322352169959, -293.5620600956856379, -317.0522711826295676 ) ) ;
#64035=CARTESIAN_POINT ( 'NONE',  ( -51.67998891948372631, -288.7385239450921972, -345.9517283624059019 ) ) ;
#64037=CARTESIAN_POINT ( 'NONE',  ( -47.57079430274748688, -293.7544940496728145, -346.0841126684085793 ) ) ;
#64038=CARTESIAN_POINT ( 'NONE',  ( -1.783228305354786603, -284.9310473934086758, -205.6351137785605658 ) ) ;
#64039=CARTESIAN_POINT ( 'NONE',  ( -68.33817933045455106, -293.5010254382592052, -202.8928401261020440 ) ) ;
#64040=CARTESIAN_POINT ( 'NONE',  ( -27.72710760521565376, -284.6563443067515209, -197.2976704723051569 ) ) ;
#64041=CARTESIAN_POINT ( 'NONE',  ( -7.034914135984592143, -283.9611432629989167, -337.3282096492065989 ) ) ;
#64043=CARTESIAN_POINT ( 'NONE',  ( -86.37198769585229741, -292.3321923883326008, -211.2255915447739483 ) ) ;
#64045=CARTESIAN_POINT ( 'NONE',  ( 33.17132662052006253, -281.7914566761671153, -251.1847165259451629 ) ) ;
#64046=CARTESIAN_POINT ( 'NONE',  ( -13.91812492433534842, -293.5497350752999068, -343.2949567851319443 ) ) ;
#64047=CARTESIAN_POINT ( 'NONE',  ( 36.23373874178597021, -288.6341432698250173, -292.5611506483164703 ) ) ;
#64048=CARTESIAN_POINT ( 'NONE',  ( -40.33008639354127212, -289.5810883632068453, -347.2545928553726640 ) ) ;
#64049=CARTESIAN_POINT ( 'NONE',  ( 23.51067020293623244, -288.2786349373474195, -310.7075053992594462 ) ) ;
#64052=CARTESIAN_POINT ( 'NONE',  ( 24.71674628524373674, -295.9968793596246428, -313.8470264043663747 ) ) ;
#64054=CARTESIAN_POINT ( 'NONE',  ( -111.1418765721582389, -295.4934666835799248, -249.9954375051690931 ) ) ;
#64055=CARTESIAN_POINT ( 'NONE',  ( -92.91297942904134288, -276.9339945138503367, -318.0606081844316577 ) ) ;
#64056=CARTESIAN_POINT ( 'NONE',  ( -67.50573499266110389, -273.1745731492483173, -199.5821811154191039 ) ) ;
#64057=CARTESIAN_POINT ( 'NONE',  ( -50.61490697035502251, -293.7046267835437448, -342.8492530863629781 ) ) ;
#64058=CARTESIAN_POINT ( 'NONE',  ( 27.51382453650762372, -276.8305632108537679, -234.5929674519288142 ) ) ;
#64059=CARTESIAN_POINT ( 'NONE',  ( 9.759455282733700443, -296.8894988464056723, -196.3621327438673347 ) ) ;
#64060=CARTESIAN_POINT ( 'NONE',  ( -45.11762753652972435, -296.3577559014474900, -343.3958771987321938 ) ) ;
#64061=CARTESIAN_POINT ( 'NONE',  ( -97.42888997956573860, -297.0486816243500243, -312.3582094261772113 ) ) ;
#64063=CARTESIAN_POINT ( 'NONE',  ( -30.64079257569892789, -296.5688866449104921, -346.2659152823010800 ) ) ;
#64065=CARTESIAN_POINT ( 'NONE',  ( -109.8309105504848588, -294.2968592590907519, -290.2443471237517656 ) ) ;
#64066=CARTESIAN_POINT ( 'NONE',  ( -36.19461568192025425, -298.7175698476569892, -193.4629270313071174 ) ) ;
#64067=CARTESIAN_POINT ( 'NONE',  ( -110.9567690822490391, -289.1521649065282986, -268.4283185786113108 ) ) ;
#64068=CARTESIAN_POINT ( 'NONE',  ( -100.9908986399047706, -275.0852220119529079, -230.6902196267084832 ) ) ;
#64069=CARTESIAN_POINT ( 'NONE',  ( -94.10410378094181283, -273.7516478925962815, -218.4036583419192823 ) ) ;
#64070=CARTESIAN_POINT ( 'NONE',  ( -110.1199159360397459, -296.7991256590588591, -276.9057601707949061 ) ) ;
#64071=CARTESIAN_POINT ( 'NONE',  ( -17.45094494918996020, -282.2874648003502216, -197.6784882941391004 ) ) ;
#64072=CARTESIAN_POINT ( 'NONE',  ( -7.712410511587266093, -279.1172581008897851, -199.8103649508600768 ) ) ;
#64074=CARTESIAN_POINT ( 'NONE',  ( -24.55870517756808624, -282.2418420497596685, -346.2433080362148985 ) ) ;
#64075=CARTESIAN_POINT ( 'NONE',  ( 39.60530611315584792, -274.9109805147836596, -271.1788498611365981 ) ) ;
#64076=CARTESIAN_POINT ( 'NONE',  ( 36.21813101987581973, -279.6998352095608880, -250.4271280434108746 ) ) ;
#64077=CARTESIAN_POINT ( 'NONE',  ( -94.49484596136692005, -277.2268040602398855, -221.5197803589919374 ) ) ;
#64078=CARTESIAN_POINT ( 'NONE',  ( -33.99587345615407230, -272.6697835427397649, -196.8479874408589581 ) ) ;
#64079=CARTESIAN_POINT ( 'NONE',  ( 34.28744386409212552, -277.2636364680579959, -247.9591903884178805 ) ) ;
#64082=CARTESIAN_POINT ( 'NONE',  ( -112.7495695017638297, -271.0950597997922387, -259.0431613161582050 ) ) ;
#64083=CARTESIAN_POINT ( 'NONE',  ( -50.25907620316200308, -289.9081487786675098, -196.1213160197946195 ) ) ;
#64084=CARTESIAN_POINT ( 'NONE',  ( -61.68858096559480231, -291.7444573679159134, -197.2554614762791800 ) ) ;
#64085=CARTESIAN_POINT ( 'NONE',  ( 36.38915228898011378, -277.7396327998554852, -284.9826716471279724 ) ) ;
#64086=CARTESIAN_POINT ( 'NONE',  ( 29.65909608989104029, -273.1067905970684251, -236.6580921268214013 ) ) ;
#64088=CARTESIAN_POINT ( 'NONE',  ( -34.50802493472657062, -284.9369429686649937, -345.8679685675796804 ) ) ;
#64089=( NAMED_UNIT ( * ) PLANE_ANGLE_UNIT ( ) SI_UNIT ( $, .RADIAN. ) );
#64090=CARTESIAN_POINT ( 'NONE',  ( -16.85317983714815782, -284.3164602854000123, -198.1605061003254491 ) ) ;
#64092=CARTESIAN_POINT ( 'NONE',  ( 28.74543454758475036, -292.7782742620349836, -302.4097828290336452 ) ) ;
#64093=CARTESIAN_POINT ( 'NONE',  ( -10.27795049251010440, -284.5487136744127383, -201.2212522984016516 ) ) ;
#64095=CARTESIAN_POINT ( 'NONE',  ( -68.13914373595406460, -293.4563744259562554, -338.7602745174829693 ) ) ;
#64096=CARTESIAN_POINT ( 'NONE',  ( -109.3168021589384580, -283.3546573709051586, -245.0176288876326964 ) ) ;
#64097=CARTESIAN_POINT ( 'NONE',  ( -96.26263673611968841, -280.7699506527359858, -225.9018216441143636 ) ) ;
#64098=CARTESIAN_POINT ( 'NONE',  ( -75.92008999479128306, -286.7543915711464138, -204.1206009370356185 ) ) ;
#64099=CARTESIAN_POINT ( 'NONE',  ( 21.72128077065429252, -280.4418637209396366, -318.1889431672349247 ) ) ;
#64100=CARTESIAN_POINT ( 'NONE',  ( 18.66176132030001966, -286.8873174291267105, -223.5163052786766116 ) ) ;
#64101=CIRCLE ( 'NONE', #61033, 1.895975569037589015 ) ;
#64102=CARTESIAN_POINT ( 'NONE',  ( -87.48386711921313008, -279.1938344061942985, -324.2233311327559022 ) ) ;
#64103=CARTESIAN_POINT ( 'NONE',  ( -109.1999551214033346, -279.1731650636668860, -284.1747338502843832 ) ) ;
#64105=CARTESIAN_POINT ( 'NONE',  ( -101.1396447034011459, -287.0686075209389401, -230.2583865339261706 ) ) ;
#64108=CARTESIAN_POINT ( 'NONE',  ( 76.38888381899823798, -299.2725563385990313, -193.3641481775453030 ) ) ;
#64109=CARTESIAN_POINT ( 'NONE',  ( -45.51812760638178901, -291.1361767615164808, -344.5567569070808531 ) ) ;
#64111=CARTESIAN_POINT ( 'NONE',  ( -37.37352853689063181, -288.5519495502701375, -190.3611179825600175 ) ) ;
#64113=CARTESIAN_POINT ( 'NONE',  ( -8.373007603888428463, -272.4302129317083541, -200.9456157213863889 ) ) ;
#64115=CARTESIAN_POINT ( 'NONE',  ( 38.43290177078794301, -291.8442865830637629, -261.8358771370611180 ) ) ;
#64116=CARTESIAN_POINT ( 'NONE',  ( -106.3999656180249787, -272.2191569659897823, -246.3851167392122363 ) ) ;
#64118=CARTESIAN_POINT ( 'NONE',  ( 26.96301397165637681, -288.5832952640606663, -234.2621550006503810 ) ) ;
#64120=CARTESIAN_POINT ( 'NONE',  ( -35.66196617530688684, -281.8336211531368463, -196.3542691956220665 ) ) ;
#64121=CARTESIAN_POINT ( 'NONE',  ( -20.60763271351048687, -290.2667648619270722, -344.9712368994705116 ) ) ;
#64122=CARTESIAN_POINT ( 'NONE',  ( -51.57702298160149468, -290.5457542013245984, -345.5319491256747710 ) ) ;
#64123=CARTESIAN_POINT ( 'NONE',  ( -94.94216819528982398, -285.8888655504377425, -318.3943016243790680 ) ) ;
#64124=CARTESIAN_POINT ( 'NONE',  ( -108.5134651390332579, -279.0923283651503084, -240.9743884994499012 ) ) ;
#64126=CARTESIAN_POINT ( 'NONE',  ( 25.30393350620322934, -292.1992669785503267, -312.6084703810788596 ) ) ;
#64127=CARTESIAN_POINT ( 'NONE',  ( 23.74860176744353879, -280.7600081435238621, -223.4676775841971335 ) ) ;
#64129=CARTESIAN_POINT ( 'NONE',  ( -49.09395476328017338, -275.7613928792315505, -197.0100318913119395 ) ) ;
#64131=CARTESIAN_POINT ( 'NONE',  ( 27.36219212280431989, -284.4805209788416391, -301.4846348637938149 ) ) ;
#64132=CARTESIAN_POINT ( 'NONE',  ( 0.5223785719801525840, -274.7950237270176217, -336.3016355121197307 ) ) ;
#64134=CARTESIAN_POINT ( 'NONE',  ( 34.39586063615828948, -280.8764366924675073, -256.4492124749717732 ) ) ;
#64136=CARTESIAN_POINT ( 'NONE',  ( -35.70453050172395848, -278.2371448505144258, -346.9596057014061898 ) ) ;
#64137=CARTESIAN_POINT ( 'NONE',  ( -95.01002813568375416, -274.5058871928542317, -224.8022832246770406 ) ) ;
#64138=CARTESIAN_POINT ( 'NONE',  ( -63.11113020456068767, -284.7833028981650045, -198.0509756357190270 ) ) ;
#64139=CARTESIAN_POINT ( 'NONE',  ( -109.4193708314066527, -292.5318094380201615, -253.4896129621295131 ) ) ;
#64140=CARTESIAN_POINT ( 'NONE',  ( -111.0497545917288562, -274.3990843985011452, -250.8311926227954700 ) ) ;
#64141=CARTESIAN_POINT ( 'NONE',  ( -18.68653884735005377, -275.6025648677230038, -196.1088475022184241 ) ) ;
#64143=CARTESIAN_POINT ( 'NONE',  ( -38.34187344849005541, -297.0648776316222666, -345.1877715485082945 ) ) ;
#64144=CARTESIAN_POINT ( 'NONE',  ( -81.73367015924681311, -281.6575907616522727, -330.6699517919837490 ) ) ;
#64145=CARTESIAN_POINT ( 'NONE',  ( -112.5455963616639821, -290.0132706360507768, -286.7963935490153062 ) ) ;
#64146=CARTESIAN_POINT ( 'NONE',  ( 16.65362924848868076, -272.8445629385341817, -218.7464661296594386 ) ) ;
#64147=CARTESIAN_POINT ( 'NONE',  ( -23.94677231391226258, -287.8205023179548903, -195.2940260259423724 ) ) ;
#64148=CARTESIAN_POINT ( 'NONE',  ( -64.17199378851334757, -290.6140415434508100, -202.1246483527534394 ) ) ;
#64150=CARTESIAN_POINT ( 'NONE',  ( -113.6636412024419371, -289.0804598119637490, -274.0445405853442935 ) ) ;
#64151=CARTESIAN_POINT ( 'NONE',  ( -103.5737144329234809, -290.6337978217831051, -239.6136340562024998 ) ) ;
#64153=CARTESIAN_POINT ( 'NONE',  ( 24.44603737428095158, -288.0259312057053762, -224.9324045427470367 ) ) ;
#64154=CARTESIAN_POINT ( 'NONE',  ( -1.456138070629751091, -276.8959523008033443, -334.0132580270123412 ) ) ;
#64155=CARTESIAN_POINT ( 'NONE',  ( -66.81839121405472781, -294.3497582806576816, -341.1751028590360306 ) ) ;
#64156=CARTESIAN_POINT ( 'NONE',  ( -112.1180784621771807, -284.9782148037290312, -288.3557872313729717 ) ) ;
#64157=CARTESIAN_POINT ( 'NONE',  ( -63.19832814098982965, -286.0576305887619242, -197.8547108223011151 ) ) ;
#64158=CARTESIAN_POINT ( 'NONE',  ( -2.414817773127506673, -282.9098542242265921, -334.5018523341619812 ) ) ;
#64159=CARTESIAN_POINT ( 'NONE',  ( -95.55820914780639441, -240.1411278548074790, -341.8388433382354492 ) ) ;
#64160=CARTESIAN_POINT ( 'NONE',  ( 83.14950132131733085, 83.50475598798475119, -301.0942469162992552 ) ) ;
#64161=CARTESIAN_POINT ( 'NONE',  ( -108.4024080554443685, -263.9389858668760098, -305.3879311740210483 ) ) ;
#64163=CARTESIAN_POINT ( 'NONE',  ( 94.64983258005516120, -299.0959783674220489, -197.2743889382824136 ) ) ;
#64164=CARTESIAN_POINT ( 'NONE',  ( 3.111926770055553515, -273.5295774831445215, -209.1634642982251648 ) ) ;
#64165=CARTESIAN_POINT ( 'NONE',  ( -56.06138294541747058, -294.7946736442961537, -344.9875233514065940 ) ) ;
#64166=CARTESIAN_POINT ( 'NONE',  ( 189.9032515046773426, 267.9733876889036992, -137.7336960540900179 ) ) ;
#64167=CARTESIAN_POINT ( 'NONE',  ( 11.48393226028832537, -273.3975359398546630, -211.3910257787479736 ) ) ;
#64168=CARTESIAN_POINT ( 'NONE',  ( -90.95405900927855214, -299.1418721902680318, -218.9398833114676108 ) ) ;
#64169=CARTESIAN_POINT ( 'NONE',  ( 14.44265908629642503, -289.6200214537574880, -322.5111287044948085 ) ) ;
#64170=CARTESIAN_POINT ( 'NONE',  ( -94.54069347392442069, -292.2773046407779702, -224.4881264791785043 ) ) ;
#64172=CARTESIAN_POINT ( 'NONE',  ( -111.3982813257405553, -297.7495281497535871, -249.9546102785856192 ) ) ;
#64173=CARTESIAN_POINT ( 'NONE',  ( 25.75235456114296184, -288.5509133476144257, -307.3003775568747642 ) ) ;
#64174=CARTESIAN_POINT ( 'NONE',  ( -8.439268677859162793, -295.4862593265058877, -341.6130484505632126 ) ) ;
#64175=CARTESIAN_POINT ( 'NONE',  ( -24.91157101875893787, -295.3901541695384481, -346.3428619613575847 ) ) ;
#64176=CARTESIAN_POINT ( 'NONE',  ( 6.674552539915903360, -292.8366658984132300, -212.1239347956079655 ) ) ;
#64178=CARTESIAN_POINT ( 'NONE',  ( 4.053434315715206182, -276.5248458520289887, -207.0870505141138551 ) ) ;
#64180=CARTESIAN_POINT ( 'NONE',  ( -113.1747728713155681, -278.2224583963825353, -257.3660426985651384 ) ) ;
#64182=CARTESIAN_POINT ( 'NONE',  ( 23.24025661270209042, -275.9227109005238390, -229.1896928347936750 ) ) ;
#64183=CARTESIAN_POINT ( 'NONE',  ( -38.36652684107135514, -275.7996055204619097, -194.3813591825203844 ) ) ;
#64184=CARTESIAN_POINT ( 'NONE',  ( -2.256388939355643330, -274.6102226422161152, -337.0501556438189823 ) ) ;
#64185=CARTESIAN_POINT ( 'NONE',  ( -110.4764251979117944, -297.2249395151284261, -268.7389001083938638 ) ) ;
#64186=CARTESIAN_POINT ( 'NONE',  ( -109.6210102986301251, -295.3086423271090553, -256.4710576432662492 ) ) ;
#64188=CARTESIAN_POINT ( 'NONE',  ( -112.7320693007894477, -278.8514755870729118, -285.7826048526360410 ) ) ;
#64189=CARTESIAN_POINT ( 'NONE',  ( -51.27880630789400840, -277.4020189159596725, -342.0183372686629468 ) ) ;
#64192=CARTESIAN_POINT ( 'NONE',  ( -4.967305565061796990, -285.1543945540529990, -201.0415907810293277 ) ) ;
#64193=CARTESIAN_POINT ( 'NONE',  ( -111.1060785622191105, -274.7299603217629738, -256.5254225831626513 ) ) ;
#64194=CARTESIAN_POINT ( 'NONE',  ( 82.67382771687083221, -297.5965108451826495, -196.9258814007443164 ) ) ;
#64196=CARTESIAN_POINT ( 'NONE',  ( 35.15758019924837896, -286.6151680731373972, -260.1694962532299655 ) ) ;
#64198=CARTESIAN_POINT ( 'NONE',  ( -54.70912216946552320, -278.0658703971398040, -198.3613683552276825 ) ) ;
#64199=CARTESIAN_POINT ( 'NONE',  ( -104.9765451648991217, -277.5133190422906182, -241.3627964370480754 ) ) ;
#64200=CARTESIAN_POINT ( 'NONE',  ( -112.1687648118101777, -286.6267572425494450, -264.5634801422433497 ) ) ;
#64201=CARTESIAN_POINT ( 'NONE',  ( -36.44601420421265203, -278.2457939693624098, -343.7652617077954460 ) ) ;
#64204=CARTESIAN_POINT ( 'NONE',  ( -14.91050453446275981, -275.0054705135414110, -343.0165856159265445 ) ) ;
#64205=CARTESIAN_POINT ( 'NONE',  ( -35.39591681071548379, -274.7285963412398360, -197.2725621310013366 ) ) ;
#64206=CARTESIAN_POINT ( 'NONE',  ( 21.97232724543506421, -284.1843652723520677, -316.5541535020900028 ) ) ;
#64208=CARTESIAN_POINT ( 'NONE',  ( -34.69235685029834571, -290.9392521634806599, -345.8746610110567872 ) ) ;
#64209=CARTESIAN_POINT ( 'NONE',  ( -41.33907348793265157, -290.0016848261755626, -195.4550004045474338 ) ) ;
#64211=CARTESIAN_POINT ( 'NONE',  ( 82.16888074921301666, -297.9818618066009321, -196.6132423200940309 ) ) ;
#64212=CARTESIAN_POINT ( 'NONE',  ( -65.99003948167957390, -272.3540516583252611, -202.6816075593507378 ) ) ;
#64213=CARTESIAN_POINT ( 'NONE',  ( 5.231080707489677906, -290.7739821697912816, -209.4834224960733025 ) ) ;
#64214=CARTESIAN_POINT ( 'NONE',  ( 5.045406874201050940, -57.93311274753654061, -355.0152878038887820 ) ) ;
#64215=CARTESIAN_POINT ( 'NONE',  ( -84.74921204074180991, -288.1716340090512745, -330.2218208164943576 ) ) ;
#64216=CARTESIAN_POINT ( 'NONE',  ( -102.4677188092241948, -285.6830467179824495, -305.1835442133593119 ) ) ;
#64217=CARTESIAN_POINT ( 'NONE',  ( 37.29907017803776625, -285.6115715254599081, -256.1228096611766318 ) ) ;
#64218=CARTESIAN_POINT ( 'NONE',  ( -70.46400878843198257, -284.9228875084473316, -336.0888868238830014 ) ) ;
#64219=CARTESIAN_POINT ( 'NONE',  ( -38.87824176622038408, -283.8747153740139311, -343.5189766448566502 ) ) ;
#64221=CARTESIAN_POINT ( 'NONE',  ( -58.50150318363142787, -293.7597959895502981, -198.0377501480702733 ) ) ;
#64222=CARTESIAN_POINT ( 'NONE',  ( 31.25621102938738716, -273.2175486719318656, -238.5561439389797158 ) ) ;
#64223=CARTESIAN_POINT ( 'NONE',  ( -27.00356244762539148, -274.5133106973700592, -194.0262031553308191 ) ) ;
#64224=CARTESIAN_POINT ( 'NONE',  ( -105.9426017625730765, -289.0463512551486360, -238.5627326758650781 ) ) ;
#64225=CARTESIAN_POINT ( 'NONE',  ( -14.58969424671998993, -276.7653283119158232, -343.9787966223019566 ) ) ;
#64226=CARTESIAN_POINT ( 'NONE',  ( -7.303795217128174144, -296.6361658221218249, -338.7092637295635313 ) ) ;
#64228=CARTESIAN_POINT ( 'NONE',  ( -110.4542110544635705, -298.8376638359844719, -287.0812184334320705 ) ) ;
#64229=CARTESIAN_POINT ( 'NONE',  ( -104.5711279879627256, -282.8401187109731154, -300.0502996197664629 ) ) ;
#64230=CARTESIAN_POINT ( 'NONE',  ( -42.27245524331343773, -277.9898048301911331, -195.5233714658876067 ) ) ;
#64232=CARTESIAN_POINT ( 'NONE',  ( -109.4403766833796396, -271.3499589852424947, -245.3713482571579618 ) ) ;
#64233=CARTESIAN_POINT ( 'NONE',  ( -103.2264729059779853, -277.4714475034114116, -302.1498597302763187 ) ) ;
#64234=CARTESIAN_POINT ( 'NONE',  ( 18.99422663204113348, -294.4036296195081377, -222.8535279554371300 ) ) ;
#64235=CARTESIAN_POINT ( 'NONE',  ( -17.06045176701547206, -279.2283937203210940, -196.4005644837530440 ) ) ;
#64236=CARTESIAN_POINT ( 'NONE',  ( 30.80890949115166677, -294.8524572014763407, -297.3122901895367249 ) ) ;
#64237=CARTESIAN_POINT ( 'NONE',  ( -81.57285785805777323, -296.9550445901002718, -332.8509930598797268 ) ) ;
#64238=CARTESIAN_POINT ( 'NONE',  ( -70.46565135321603179, -297.4361464178937808, -205.2948902160746911 ) ) ;
#64239=CARTESIAN_POINT ( 'NONE',  ( -42.78430026052969737, -291.1208601633182411, -345.2153724069146392 ) ) ;
#64240=CARTESIAN_POINT ( 'NONE',  ( -89.88779501488360779, -285.5016321290386259, -214.0044260576217710 ) ) ;
#64241=CARTESIAN_POINT ( 'NONE',  ( -55.02201972861390544, -271.9667315955380218, -196.6881122300655136 ) ) ;
#64242=CARTESIAN_POINT ( 'NONE',  ( 35.84969678633999735, -287.0826467082037539, -246.2736572080849839 ) ) ;
#64243=CARTESIAN_POINT ( 'NONE',  ( -109.2085981721099159, -280.7933829587623791, -250.1395495399056301 ) ) ;
#64245=CARTESIAN_POINT ( 'NONE',  ( -10.65309267712260777, -285.4677292894647280, -202.1483782838506613 ) ) ;
#64246=CARTESIAN_POINT ( 'NONE',  ( -106.9519126385471424, -288.1882506219339461, -298.2791938581951854 ) ) ;
#64247=CARTESIAN_POINT ( 'NONE',  ( 85.37101130053461873, 80.99577858023421584, -298.5812782549759845 ) ) ;
#64248=CARTESIAN_POINT ( 'NONE',  ( 9.074412919876589712, -286.2172963857036621, -213.9383132758052568 ) ) ;
#64249=CARTESIAN_POINT ( 'NONE',  ( 33.35393457074724211, -282.8768350914514258, -300.4125903019410657 ) ) ;
#64251=CARTESIAN_POINT ( 'NONE',  ( -56.11959337319295571, -290.8748872662643521, -195.8737470019289333 ) ) ;
#64252=CARTESIAN_POINT ( 'NONE',  ( -90.51467456775094433, -280.9146923019625888, -215.7066333863451746 ) ) ;
#64253=CARTESIAN_POINT ( 'NONE',  ( -104.3696486666726599, -280.3481382597793186, -233.4754515755964519 ) ) ;
#64254=CARTESIAN_POINT ( 'NONE',  ( 35.51999108845736686, -281.3262201609597355, -265.8695750903006001 ) ) ;
#64255=CARTESIAN_POINT ( 'NONE',  ( 24.69264436449613243, -276.9814485151051713, -228.1866902967092869 ) ) ;
#64256=CARTESIAN_POINT ( 'NONE',  ( 19.52968153547678298, -294.2585922463209727, -322.3487600808773550 ) ) ;
#64257=CARTESIAN_POINT ( 'NONE',  ( 8.981391797661739673, -286.4329754034737334, -328.8933138579299111 ) ) ;
#64258=CARTESIAN_POINT ( 'NONE',  ( -73.07676811720180865, -293.1867500357013228, -203.0452172305451768 ) ) ;
#64259=CARTESIAN_POINT ( 'NONE',  ( -90.25951223309061788, -296.2022589853284558, -219.5545602154507776 ) ) ;
#64261=CARTESIAN_POINT ( 'NONE',  ( -51.26369735830706276, -285.1515284000663542, -343.5402582968472984 ) ) ;
#64262=CARTESIAN_POINT ( 'NONE',  ( -98.75338481821634673, -295.6711950852856603, -309.9593555270666911 ) ) ;
#64263=CARTESIAN_POINT ( 'NONE',  ( -2.209742686731688277, -293.5857512618093210, -202.1757467171505880 ) ) ;
#64265=CARTESIAN_POINT ( 'NONE',  ( -2.372615935219600125, -283.2279348621967188, -334.5708781241722818 ) ) ;
#64266=CARTESIAN_POINT ( 'NONE',  ( 26.74075959475894138, -274.0534428312576551, -228.0969656936518390 ) ) ;
#64267=CARTESIAN_POINT ( 'NONE',  ( -65.40208670600769381, -290.0607710452212586, -342.0129663199547281 ) ) ;
#64268=CARTESIAN_POINT ( 'NONE',  ( -108.1570458389323903, -282.3435728532241455, -297.4423969224559414 ) ) ;
#64269=CARTESIAN_POINT ( 'NONE',  ( -100.6607907529931083, -290.3071342874925449, -314.1382473307544956 ) ) ;
#64270=CARTESIAN_POINT ( 'NONE',  ( 33.72991039674568725, -287.6636870339884240, -253.5466128749491759 ) ) ;
#64272=CARTESIAN_POINT ( 'NONE',  ( 202.2090562182569613, 292.1033822784109475, -53.99999999998392042 ) ) ;
#64273=CARTESIAN_POINT ( 'NONE',  ( -95.95921662488163406, -276.6952119285918457, -223.5744983911110353 ) ) ;
#64274=CARTESIAN_POINT ( 'NONE',  ( -83.53178740183430762, -278.5972817326481277, -213.5586391358351932 ) ) ;
#64276=CARTESIAN_POINT ( 'NONE',  ( 2.885043427152404583, -279.5260208023804580, -209.0136983235933030 ) ) ;
#64277=CARTESIAN_POINT ( 'NONE',  ( 39.53348774345503358, -275.1573764929423760, -265.4453586957677658 ) ) ;
#64278=CARTESIAN_POINT ( 'NONE',  ( 175.3651808782167620, 240.6162257589489286, -178.0254516555434350 ) ) ;
#64279=CARTESIAN_POINT ( 'NONE',  ( -33.92333132851602073, -278.6691002554712213, -194.0268461996747931 ) ) ;
#64280=CARTESIAN_POINT ( 'NONE',  ( -56.77077590340982738, -281.3240102541504370, -342.4330113552243233 ) ) ;
#64281=CARTESIAN_POINT ( 'NONE',  ( -111.6099308129362129, -298.1086455285047805, -286.4298431388921244 ) ) ;
#64283=CARTESIAN_POINT ( 'NONE',  ( 35.59567580923845043, -293.9778711251062759, -265.3058431170756535 ) ) ;
#64285=CARTESIAN_POINT ( 'NONE',  ( -84.13019986963037411, -290.0778094746079319, -213.6859049832245034 ) ) ;
#64286=CARTESIAN_POINT ( 'NONE',  ( -44.04215518520750550, -274.6210908728622826, -193.7022882765053566 ) ) ;
#64287=CARTESIAN_POINT ( 'NONE',  ( -35.14989057605235701, -298.2470232487723933, -197.3610538051364642 ) ) ;
#64293=CARTESIAN_POINT ( 'NONE',  ( 29.24772827788807561, -282.2184733024449201, -239.5788855332017704 ) ) ;
#64294=CARTESIAN_POINT ( 'NONE',  ( -25.57490725043009050, -281.9602612998589848, -195.2910400742656805 ) ) ;
#64295=CARTESIAN_POINT ( 'NONE',  ( -103.2295756950217367, -283.1780771136274666, -302.4494280215002391 ) ) ;
#64296=CARTESIAN_POINT ( 'NONE',  ( -24.68876554313450811, -282.0757311310477462, -197.2121690888495777 ) ) ;
#64297=CARTESIAN_POINT ( 'NONE',  ( 36.28074556067961964, -273.9765777567299665, -266.1181661493768047 ) ) ;
#64298=CARTESIAN_POINT ( 'NONE',  ( 82.64890176555634582, -299.5541904835127980, -197.7582414438974183 ) ) ;
#64301=CARTESIAN_POINT ( 'NONE',  ( -62.34376567437308836, -278.1719733601764801, -343.0744146994452990 ) ) ;
#64305=CARTESIAN_POINT ( 'NONE',  ( -110.6137667434262681, -286.3064784948170427, -288.0114343624215394 ) ) ;
#64307=CARTESIAN_POINT ( 'NONE',  ( 35.69658172111954286, -292.6828998638386565, -265.3153683164657650 ) ) ;
#64308=CARTESIAN_POINT ( 'NONE',  ( 21.40577683879840620, -287.5701198435004358, -319.9801338632363468 ) ) ;
#64309=CARTESIAN_POINT ( 'NONE',  ( -37.25752343330825056, -284.2930418577966520, -196.3352183213253284 ) ) ;
#64310=CARTESIAN_POINT ( 'NONE',  ( -110.8153276975776009, -283.1916945597094468, -265.4076021161958465 ) ) ;
#64311=CARTESIAN_POINT ( 'NONE',  ( -23.61897982175615951, -287.1143691806655625, -343.1435868860552887 ) ) ;
#64312=CARTESIAN_POINT ( 'NONE',  ( -4.636520057316280585, -283.8164013608051732, -336.0688169426838954 ) ) ;
#64313=CARTESIAN_POINT ( 'NONE',  ( -19.01341392722402546, -272.2877638636493316, -197.5814888809499905 ) ) ;
#64314=CARTESIAN_POINT ( 'NONE',  ( -73.21815181915705750, -283.9848573080953997, -203.0767914262243039 ) ) ;
#64315=CARTESIAN_POINT ( 'NONE',  ( -67.40060577870521286, -297.4465505687067548, -339.0740195548497127 ) ) ;
#64316=CARTESIAN_POINT ( 'NONE',  ( -105.0171709743313926, -282.9819557775090288, -237.6493606287095588 ) ) ;
#64317=CARTESIAN_POINT ( 'NONE',  ( -96.60313430386329969, -280.0936449559250150, -227.3321641490323657 ) ) ;
#64318=CARTESIAN_POINT ( 'NONE',  ( 35.92673468165072848, -289.3365992374277198, -253.5182266915477669 ) ) ;
#64321=CARTESIAN_POINT ( 'NONE',  ( 36.35134775167517063, -295.2588896797203120, -253.6104121694705498 ) ) ;
#64322=CARTESIAN_POINT ( 'NONE',  ( -51.68772512496835247, -275.2355271519058988, -343.9762809082972126 ) ) ;
#64323=CARTESIAN_POINT ( 'NONE',  ( -74.59164692859015133, -290.7666187596316263, -203.1554613454208038 ) ) ;
#64324=CARTESIAN_POINT ( 'NONE',  ( -72.52370616124974845, -293.9258837640778097, -335.2497840450249100 ) ) ;
#64325=CARTESIAN_POINT ( 'NONE',  ( -103.8087499645918399, -277.6592795817295496, -238.8827533835867030 ) ) ;
#64326=CARTESIAN_POINT ( 'NONE',  ( -35.07725289688835346, -296.2203756193097206, -196.1266373355561541 ) ) ;
#64327=CARTESIAN_POINT ( 'NONE',  ( -38.92488140263169782, -293.3470546993085009, -196.8850197163308167 ) ) ;
#64328=CARTESIAN_POINT ( 'NONE',  ( -20.19161114001083490, -279.3376638359844719, -345.3538533559490702 ) ) ;
#64329=CARTESIAN_POINT ( 'NONE',  ( -3.553361353515080090, -293.0942587454981094, -338.7938315540193912 ) ) ;
#64330=CARTESIAN_POINT ( 'NONE',  ( -42.70189713450172064, -290.7208926183793665, -344.0173623997341110 ) ) ;
#64331=CARTESIAN_POINT ( 'NONE',  ( -2.500232579277053002, -290.7463978564754825, -202.8184191527291489 ) ) ;
#64333=CARTESIAN_POINT ( 'NONE',  ( -80.74048096559134535, -291.0788983514864867, -329.8544814643549898 ) ) ;
#64335=CARTESIAN_POINT ( 'NONE',  ( -107.8787547516812708, -291.0967423015341069, -289.9674358561701411 ) ) ;
#64338=CARTESIAN_POINT ( 'NONE',  ( -112.2549087152298597, -291.9591115730350452, -254.2985499766523105 ) ) ;
#64339=CARTESIAN_POINT ( 'NONE',  ( 35.74233106217786116, -279.3375189914528960, -251.9999853570184030 ) ) ;
#64340=CARTESIAN_POINT ( 'NONE',  ( -77.25515655472437970, -291.5003627885799915, -209.2389779997480161 ) ) ;
#64341=CARTESIAN_POINT ( 'NONE',  ( -22.56617992221908509, -280.2361386073488347, -194.7377947474200255 ) ) ;
#64342=CARTESIAN_POINT ( 'NONE',  ( -16.15173329207562603, -282.4523106554419201, -344.4213171312875374 ) ) ;
#64344=CARTESIAN_POINT ( 'NONE',  ( 21.08896203919870516, -284.9047667092990537, -223.3209963924220460 ) ) ;
#64346=CARTESIAN_POINT ( 'NONE',  ( 8.539088898974560138, -280.5560889380074059, -328.7861448993861586 ) ) ;
#64347=CARTESIAN_POINT ( 'NONE',  ( -24.11297164892630818, -284.2207929268104749, -196.4841816055509298 ) ) ;
#64348=CARTESIAN_POINT ( 'NONE',  ( 8.148869718730979983, -279.1411590877679032, -209.0311129058181621 ) ) ;
#64350=CARTESIAN_POINT ( 'NONE',  ( 26.10937971688296955, -285.9020215805663838, -227.2626837416132446 ) ) ;
#64351=CARTESIAN_POINT ( 'NONE',  ( 34.32479902042874187, -276.5486664835795523, -285.0755539980270328 ) ) ;
#64353=CARTESIAN_POINT ( 'NONE',  ( -49.84408609892941655, -293.4902922642074827, -197.5759430103919101 ) ) ;
#64354=CARTESIAN_POINT ( 'NONE',  ( -18.71134374824497115, -275.7126454326285625, -196.2017478159464190 ) ) ;
#64355=CARTESIAN_POINT ( 'NONE',  ( -92.74545013234352098, -277.5418670399407688, -317.9269878085795540 ) ) ;
#64356=CARTESIAN_POINT ( 'NONE',  ( -90.78746412824945367, -291.4861909013414447, -214.8565257819194585 ) ) ;
#64357=CARTESIAN_POINT ( 'NONE',  ( 37.84263308624665711, -279.7343271825826037, -278.3902767621600560 ) ) ;
#64358=CARTESIAN_POINT ( 'NONE',  ( -39.20956439237792779, -291.8626716879232958, -193.3707413523379159 ) ) ;
#64360=CARTESIAN_POINT ( 'NONE',  ( -107.6177114222323326, -289.8831974916220702, -249.7085902318378317 ) ) ;
#64361=CARTESIAN_POINT ( 'NONE',  ( -30.79166626403450380, -292.9691785523134513, -345.0745552280749280 ) ) ;
#64362=ORIENTED_EDGE ( 'NONE', *, *, #76024, .F. ) ;
#64363=CARTESIAN_POINT ( 'NONE',  ( -22.72219127671001360, -291.7519975002983301, -198.7771923958328273 ) ) ;
#64365=CARTESIAN_POINT ( 'NONE',  ( 27.33386217378598815, -273.4809262143061233, -301.5434626090942629 ) ) ;
#64366=CARTESIAN_POINT ( 'NONE',  ( -95.38529460948660699, -296.2923134969316266, -220.0447483214486226 ) ) ;
#64367=CARTESIAN_POINT ( 'NONE',  ( -113.1085767075949491, -285.7290089238606470, -281.3497512366016053 ) ) ;
#64368=CARTESIAN_POINT ( 'NONE',  ( 35.62989344132367364, -287.4303335985832177, -273.7619457919724937 ) ) ;
#64369=CARTESIAN_POINT ( 'NONE',  ( -18.82420813340162979, -278.3294950543986488, -341.6900058248146479 ) ) ;
#64370=CARTESIAN_POINT ( 'NONE',  ( 25.80554818424433705, -292.1111315348035191, -310.2610728881064119 ) ) ;
#64371=CARTESIAN_POINT ( 'NONE',  ( -85.11532307148122811, -297.4820003728777920, -326.9585154676223056 ) ) ;
#64372=CARTESIAN_POINT ( 'NONE',  ( -1.288497971199028980, -275.3578437271847861, -334.3505975099982379 ) ) ;
#64375=CARTESIAN_POINT ( 'NONE',  ( -72.06829632172608058, -295.1655267636355688, -339.0619753893969346 ) ) ;
#64376=CARTESIAN_POINT ( 'NONE',  ( -2.674383704818851459, -290.5105819744737232, -336.2930346170012967 ) ) ;
#64377=CARTESIAN_POINT ( 'NONE',  ( 202.8433248031682865, 295.9636489450775230, -54.00000000006134115 ) ) ;
#64379=CARTESIAN_POINT ( 'NONE',  ( -45.36540959979937071, -289.8079119360440359, -343.0213736551908141 ) ) ;
#64381=CARTESIAN_POINT ( 'NONE',  ( -36.74231642350465421, -279.1182660441641019, -193.5857453234507659 ) ) ;
#64382=CARTESIAN_POINT ( 'NONE',  ( 6.562617068261710429, -295.1242884894569443, -333.5585932379202063 ) ) ;
#64383=CARTESIAN_POINT ( 'NONE',  ( -82.14164690048340844, -287.7955781288341655, -331.4616110015456911 ) ) ;
#64384=CARTESIAN_POINT ( 'NONE',  ( -113.1190505072844701, -297.0549098104040695, -256.8135181553838606 ) ) ;
#64385=CARTESIAN_POINT ( 'NONE',  ( 35.44584944960058692, -293.9624009852225299, -276.1972222645192687 ) ) ;
#64388=CARTESIAN_POINT ( 'NONE',  ( -43.11039638419920550, -290.6438594746966260, -346.4494212641529316 ) ) ;
#64389=CARTESIAN_POINT ( 'NONE',  ( -99.90806341382575795, -293.4094976428775681, -320.2154176792147382 ) ) ;
#64390=CARTESIAN_POINT ( 'NONE',  ( -95.82288174436936856, -278.5753332783679070, -220.4082995835377687 ) ) ;
#64391=CARTESIAN_POINT ( 'NONE',  ( -15.57552213279881670, -284.7699773003335508, -341.9590363857040529 ) ) ;
#64392=CARTESIAN_POINT ( 'NONE',  ( 19.85782846150384273, -285.4346281535941898, -219.6191930782352131 ) ) ;
#64393=CARTESIAN_POINT ( 'NONE',  ( 36.55072908179593583, -285.7485823849149824, -279.3735040521349333 ) ) ;
#64394=CARTESIAN_POINT ( 'NONE',  ( 31.90066331500138119, -277.8114637379513852, -301.1149890022907698 ) ) ;
#64396=CARTESIAN_POINT ( 'NONE',  ( -110.2801391741247983, -278.5126121371581007, -273.3584684002801168 ) ) ;
#64397=CARTESIAN_POINT ( 'NONE',  ( -95.68810345742923573, -278.5187732037104524, -226.2995676792914139 ) ) ;
#64398=CARTESIAN_POINT ( 'NONE',  ( -5.256162063466479850, -275.5442637721104688, -200.7047416907461184 ) ) ;
#64399=CARTESIAN_POINT ( 'NONE',  ( -112.3256842372725117, -277.5448076277122027, -254.6323289033134358 ) ) ;
#64400=CARTESIAN_POINT ( 'NONE',  ( 4.168043760347364568, -58.11863228567613504, -352.1996900385278195 ) ) ;
#64401=CARTESIAN_POINT ( 'NONE',  ( -93.00981761228777600, -274.2181319795718082, -217.4847574824377432 ) ) ;
#64402=CARTESIAN_POINT ( 'NONE',  ( -87.09248407922208912, -298.8006180069590982, -212.2959583402710848 ) ) ;
#64403=CARTESIAN_POINT ( 'NONE',  ( -106.6662871844225293, -281.4805209788417528, -237.0123917617630980 ) ) ;
#64405=CARTESIAN_POINT ( 'NONE',  ( 82.64742324267871254, -299.6703133987807632, -192.8578546138987519 ) ) ;
#64406=CARTESIAN_POINT ( 'NONE',  ( -57.49249684837443652, -286.8656650487132538, -199.8230215280137543 ) ) ;
#64407=CARTESIAN_POINT ( 'NONE',  ( -87.10348453532112956, -287.1306894329230772, -212.8654993279931205 ) ) ;
#64408=CARTESIAN_POINT ( 'NONE',  ( -5.755888562898014982, -287.9740461472354127, -336.2870550358711625 ) ) ;
#64409=CARTESIAN_POINT ( 'NONE',  ( -106.9526328098753538, -283.6397291934030704, -303.1306915871295473 ) ) ;
#64410=CARTESIAN_POINT ( 'NONE',  ( -62.56341090780811953, -278.1184138706750559, -200.9508150458516980 ) ) ;
#64411=CARTESIAN_POINT ( 'NONE',  ( -70.55599010159551199, -287.4699311427598900, -203.9566022471602196 ) ) ;
#64412=CARTESIAN_POINT ( 'NONE',  ( 17.59245306459891012, -279.3359059350454459, -221.2393655068098610 ) ) ;
#64413=CARTESIAN_POINT ( 'NONE',  ( -51.35864970847332245, -278.5503280460064843, -342.5052002146613290 ) ) ;
#64414=CARTESIAN_POINT ( 'NONE',  ( 34.90156370213900772, -275.8996708140516603, -259.3728939575050845 ) ) ;
#64415=CARTESIAN_POINT ( 'NONE',  ( -4.517197329014404517, -287.4241552041630712, -339.5893979007939265 ) ) ;
#64417=CARTESIAN_POINT ( 'NONE',  ( -58.43258919843992771, -284.1207569454701343, -344.3037986221444839 ) ) ;
#64418=CARTESIAN_POINT ( 'NONE',  ( -114.2931396907330139, -285.0133028107742916, -272.8535005684336738 ) ) ;
#64419=CARTESIAN_POINT ( 'NONE',  ( 4.921427777927685376, -280.8080200882454278, -210.8394578571337945 ) ) ;
#64422=DIRECTION ( 'NONE',  ( 0.000000000000000000, 0.000000000000000000, -1.000000000000000000 ) ) ;
#64423=CARTESIAN_POINT ( 'NONE',  ( 24.85155857719669825, -289.9946971379707179, -313.7213640003960791 ) ) ;
#64424=CARTESIAN_POINT ( 'NONE',  ( -113.6946172941926108, -289.2980369915989627, -265.5103127030022279 ) ) ;
#64425=CARTESIAN_POINT ( 'NONE',  ( -34.46170431063792705, -297.2862779787807881, -197.2000453612116928 ) ) ;
#64426=CARTESIAN_POINT ( 'NONE',  ( 38.75226698425536398, -292.7573656211983462, -258.9120952859369140 ) ) ;
#64427=CARTESIAN_POINT ( 'NONE',  ( -72.70845329467637441, -288.0094597772149996, -335.0132681701780939 ) ) ;
#64428=CARTESIAN_POINT ( 'NONE',  ( 33.30749109056069557, -292.0803484970601858, -292.4216210125902080 ) ) ;
#64429=CARTESIAN_POINT ( 'NONE',  ( 32.64762668622217490, -288.4652903822090479, -248.2142144258249914 ) ) ;
#64430=CARTESIAN_POINT ( 'NONE',  ( -85.33152481854864391, -287.9090924074130839, -210.2361428286349110 ) ) ;
#64431=CARTESIAN_POINT ( 'NONE',  ( -23.65134415127682388, -290.8774919745281409, -344.1537428290707226 ) ) ;
#64432=CARTESIAN_POINT ( 'NONE',  ( -70.07574955262866467, -289.6217537651576777, -202.6964267482321134 ) ) ;
#64433=CARTESIAN_POINT ( 'NONE',  ( -0.2695735499708724059, -294.5449217423559389, -205.1060487566341521 ) ) ;
#64434=CARTESIAN_POINT ( 'NONE',  ( -110.3292873604746944, -285.4142724016641068, -276.3794697227623374 ) ) ;
#64435=CARTESIAN_POINT ( 'NONE',  ( 22.49984862790955731, -294.9310972230312586, -224.8534924383180282 ) ) ;
#64438=CARTESIAN_POINT ( 'NONE',  ( -20.92538960612227683, -300.1762811758464977, -194.7957882766897626 ) ) ;
#64439=CARTESIAN_POINT ( 'NONE',  ( 7.885778248651064359, -281.6135021240404512, -327.9330022750591525 ) ) ;
#64440=CARTESIAN_POINT ( 'NONE',  ( -96.71493259058206604, -281.9238446246076251, -316.2058826776774936 ) ) ;
#64441=CARTESIAN_POINT ( 'NONE',  ( -96.39389576316085595, -295.0864808814266667, -319.5445441175951942 ) ) ;
#64442=CARTESIAN_POINT ( 'NONE',  ( 10.15226699601402771, -272.9569511001067781, -213.5287057410741340 ) ) ;
#64443=CARTESIAN_POINT ( 'NONE',  ( -79.46664140816740485, -275.7053703248596435, -331.7981890460020509 ) ) ;
#64444=CARTESIAN_POINT ( 'NONE',  ( -109.3646791436865584, -297.6748559057865009, -285.0502031847843796 ) ) ;
#64445=CARTESIAN_POINT ( 'NONE',  ( -68.58639436204767037, -272.2242934687376987, -200.6160999988700269 ) ) ;
#64446=CARTESIAN_POINT ( 'NONE',  ( -58.56093415721047535, -296.7572467868780564, -340.8247186789637908 ) ) ;
#64448=CARTESIAN_POINT ( 'NONE',  ( -88.24542140941591128, -298.1201237186459707, -217.7412304273850054 ) ) ;
#64450=CARTESIAN_POINT ( 'NONE',  ( 35.78687109716308612, -285.3398179259469885, -252.1781898070272803 ) ) ;
#64451=CARTESIAN_POINT ( 'NONE',  ( -90.19514101269322737, -273.1118063077031479, -219.9889447561661768 ) ) ;
#64452=CARTESIAN_POINT ( 'NONE',  ( 32.71202783455942864, -287.1421413503600775, -238.2722378208749774 ) ) ;
#64453=CARTESIAN_POINT ( 'NONE',  ( 39.33401220729152925, -287.1263292437990913, -262.9635165093593514 ) ) ;
#64454=CARTESIAN_POINT ( 'NONE',  ( 7.938366319146354044, -296.4167145600439426, -330.5950152696555051 ) ) ;
#64455=CARTESIAN_POINT ( 'NONE',  ( 20.78555917980293088, -290.9013635912927498, -223.2107013699527727 ) ) ;
#64456=CARTESIAN_POINT ( 'NONE',  ( -38.15791405499206235, -279.2393389542459659, -193.5269288731509505 ) ) ;
#64457=CARTESIAN_POINT ( 'NONE',  ( 21.31550574532286291, -284.4094976428775681, -223.6242672951989618 ) ) ;
#64458=DIRECTION ( 'NONE',  ( 0.000000000000000000, 0.000000000000000000, -1.000000000000000000 ) ) ;
#64459=CARTESIAN_POINT ( 'NONE',  ( -14.42755086092044614, -285.1507276763289269, -200.5792453577557239 ) ) ;
#64461=CARTESIAN_POINT ( 'NONE',  ( -12.65289333048296250, -286.7309927975702522, -341.1810549110675197 ) ) ;
#64462=CARTESIAN_POINT ( 'NONE',  ( -70.84878265057240299, -299.2026690299682059, -204.5920842196651961 ) ) ;
#64463=CARTESIAN_POINT ( 'NONE',  ( -70.99158755597717629, -281.0420581609740793, -201.7587027806579840 ) ) ;
#64464=CARTESIAN_POINT ( 'NONE',  ( -110.0126428132140859, -294.3171242747013707, -290.2945294859731007 ) ) ;
#64465=CARTESIAN_POINT ( 'NONE',  ( -2.428663479340355202, -282.5766268895550297, -334.4853119061081088 ) ) ;
#64466=CARTESIAN_POINT ( 'NONE',  ( -110.7991569379851455, -296.4282270007389570, -293.4920834983084319 ) ) ;
#64467=CARTESIAN_POINT ( 'NONE',  ( -92.37544196934980789, -298.7664715934879496, -221.3509658476129971 ) ) ;
#64468=CARTESIAN_POINT ( 'NONE',  ( 35.98541858618412448, -285.3995463850646956, -252.1279651401911508 ) ) ;
#64469=CARTESIAN_POINT ( 'NONE',  ( -25.73099632562329120, -282.2002419152404968, -196.2652867665148619 ) ) ;
#64470=CARTESIAN_POINT ( 'NONE',  ( -109.5970128993856036, -295.4538860901553790, -282.3017303933320363 ) ) ;
#64472=CARTESIAN_POINT ( 'NONE',  ( 202.9738562182569694, 296.4636489450776367, -53.99999999999997868 ) ) ;
#64473=CARTESIAN_POINT ( 'NONE',  ( -38.89457391577523282, -285.0515845840061502, -345.0025405317936702 ) ) ;
#64475=CARTESIAN_POINT ( 'NONE',  ( 35.78497577281001440, -284.8380690714490129, -253.7030783399848985 ) ) ;
#64476=CARTESIAN_POINT ( 'NONE',  ( -20.17215399371378481, -276.0342699359373455, -345.3114177842048207 ) ) ;
#64477=CARTESIAN_POINT ( 'NONE',  ( 18.47795866041701984, -292.7171004276331132, -223.3168229271128098 ) ) ;
#64478=CARTESIAN_POINT ( 'NONE',  ( 33.77765719712441239, -282.8190653423158096, -251.0062878782554208 ) ) ;
#64480=CARTESIAN_POINT ( 'NONE',  ( 31.02676457209103233, -277.5220762985101146, -298.2855571519621094 ) ) ;
#64481=CARTESIAN_POINT ( 'NONE',  ( 17.26732991740023948, -283.8891956746959409, -323.5806242021854473 ) ) ;
#64482=CARTESIAN_POINT ( 'NONE',  ( 32.60507000949143475, -280.6423018395626627, -292.7656843468159877 ) ) ;
#64483=CARTESIAN_POINT ( 'NONE',  ( -107.3911718099231365, -280.9023202273864968, -243.4186577055732243 ) ) ;
#64484=CARTESIAN_POINT ( 'NONE',  ( -111.0377458638795218, -273.0009844524573737, -247.8653269367185885 ) ) ;
#64485=CARTESIAN_POINT ( 'NONE',  ( -6.576650455173027154, -276.4925527313734506, -340.9622829217270805 ) ) ;
#64486=CARTESIAN_POINT ( 'NONE',  ( 19.56186268391509486, -294.8035970298693655, -222.3684233302651876 ) ) ;
#64487=FACE_OUTER_BOUND ( 'NONE', #69832, .T. ) ;
#64490=CARTESIAN_POINT ( 'NONE',  ( 23.87406316895902947, -292.2941942965364888, -315.0252725030736656 ) ) ;
#64491=CARTESIAN_POINT ( 'NONE',  ( -78.88491528544589926, -272.9832558776610654, -210.1985046608133416 ) ) ;
#64492=CARTESIAN_POINT ( 'NONE',  ( 27.52682286650468413, -295.6036830218861837, -310.6447832343832829 ) ) ;
#64493=CARTESIAN_POINT ( 'NONE',  ( 13.14571598031880839, -295.5702579669950865, -328.0424802249561935 ) ) ;
#64494=CARTESIAN_POINT ( 'NONE',  ( -83.66159047939355276, -291.6896254579139622, -329.1360801790992809 ) ) ;
#64495=CARTESIAN_POINT ( 'NONE',  ( -110.2787489673270755, -276.3358494421663636, -287.1576229926963038 ) ) ;
#64496=CARTESIAN_POINT ( 'NONE',  ( -26.79376929207654712, -278.8371176923062649, -344.0500272637839316 ) ) ;
#64497=CARTESIAN_POINT ( 'NONE',  ( -0.05748086624716639004, -292.6321896449697419, -334.8497560416354304 ) ) ;
#64498=CARTESIAN_POINT ( 'NONE',  ( 21.89451022196698915, -282.7695589643986978, -223.1030490473544319 ) ) ;
#64499=CARTESIAN_POINT ( 'NONE',  ( -108.6630568638028365, -283.6958636808075198, -253.3515641638277600 ) ) ;
#64500=CARTESIAN_POINT ( 'NONE',  ( 169.7216216461204112, 230.9133231598102043, -192.0398292467810677 ) ) ;
#64502=CARTESIAN_POINT ( 'NONE',  ( 1.108834432361260003, -282.1904798437578847, -332.4978837284465953 ) ) ;
#64503=CARTESIAN_POINT ( 'NONE',  ( 8.351297179918017122, -281.7405340506363700, -208.7025609395122672 ) ) ;
#64504=CARTESIAN_POINT ( 'NONE',  ( -102.1742072254386500, -283.8841529935455128, -229.5597118603892284 ) ) ;
#64505=CARTESIAN_POINT ( 'NONE',  ( -64.66980700518718095, -280.6452912524573549, -198.5694668202752382 ) ) ;
#64507=CARTESIAN_POINT ( 'NONE',  ( -112.1103476709528053, -279.8790841208067377, -285.6688771612105597 ) ) ;
#64508=CARTESIAN_POINT ( 'NONE',  ( 27.36219212280431989, -296.4805209788416391, -301.4846348637938149 ) ) ;
#64511=CARTESIAN_POINT ( 'NONE',  ( -85.37473520293464446, -299.3889410144918770, -212.6926992077347620 ) ) ;
#64512=CARTESIAN_POINT ( 'NONE',  ( -102.2294517245494205, -277.0664893436626244, -233.4636046099098792 ) ) ;
#64513=CARTESIAN_POINT ( 'NONE',  ( -112.3560681319127781, -292.1587307900924202, -282.4779908182102304 ) ) ;
#64514=CARTESIAN_POINT ( 'NONE',  ( 30.67736333966619000, -293.2600484201256563, -297.2820263624678319 ) ) ;
#64515=CARTESIAN_POINT ( 'NONE',  ( -40.34264086357487855, -288.5965531143997964, -347.2541037017051053 ) ) ;
#64517=CARTESIAN_POINT ( 'NONE',  ( 23.54835874479473645, -292.7466679036244273, -316.5239496233062937 ) ) ;
#64518=CARTESIAN_POINT ( 'NONE',  ( -41.34618498889668103, -284.4007977450286830, -196.6572040888442530 ) ) ;
#64519=CARTESIAN_POINT ( 'NONE',  ( -6.783065363192309682, -294.3180397001498818, -202.7073278129387859 ) ) ;
#64520=CARTESIAN_POINT ( 'NONE',  ( -4.266184045978813622, -284.9762626408649453, -204.5073558250194310 ) ) ;
#64521=CARTESIAN_POINT ( 'NONE',  ( -65.48918402116464677, -284.7432030361666762, -338.2641479230591131 ) ) ;
#64523=CARTESIAN_POINT ( 'NONE',  ( -74.57529698846450117, -292.5104216721237549, -203.2308008520193710 ) ) ;
#64524=CARTESIAN_POINT ( 'NONE',  ( 23.73052652282639130, -281.4878865413351150, -230.1678779353851780 ) ) ;
#64525=CARTESIAN_POINT ( 'NONE',  ( 30.54333382965190680, -292.8073581242786645, -305.8523969403868250 ) ) ;
#64526=CARTESIAN_POINT ( 'NONE',  ( 36.99080631240903472, -288.5991287849770401, -289.8248613851279742 ) ) ;
#64527=CARTESIAN_POINT ( 'NONE',  ( -31.82492592540377174, -289.4767734014784537, -347.1540520971149135 ) ) ;
#64528=CARTESIAN_POINT ( 'NONE',  ( -42.67624737291180992, -286.1496899679098647, -197.5436669105693284 ) ) ;
#64529=VERTEX_POINT ( 'NONE', #73457 ) ;
#64531=CARTESIAN_POINT ( 'NONE',  ( 36.86565793160876581, -295.6068153806737087, -285.6442293638363026 ) ) ;
#64532=CARTESIAN_POINT ( 'NONE',  ( -48.87897920895333925, -296.5931000476635973, -194.6758622879561358 ) ) ;
#64533=CARTESIAN_POINT ( 'NONE',  ( -99.38077421114850551, -277.0740926879548169, -309.3732386908070566 ) ) ;
#64534=CARTESIAN_POINT ( 'NONE',  ( -97.76084207921024927, -272.6974328686652598, -222.7265277202310187 ) ) ;
#64535=CARTESIAN_POINT ( 'NONE',  ( 4.191335080983512817, -292.9608134091878355, -331.2357000134188638 ) ) ;
#64536=CARTESIAN_POINT ( 'NONE',  ( 14.45630348962820122, -278.0719816276331358, -323.2997177924704033 ) ) ;
#64537=CARTESIAN_POINT ( 'NONE',  ( -110.8016007932268963, -270.8350927823201459, -259.3097206377961470 ) ) ;
#64538=CARTESIAN_POINT ( 'NONE',  ( 22.11741417325055181, -294.1582104793656072, -227.3078537129923689 ) ) ;
#64539=CARTESIAN_POINT ( 'NONE',  ( -108.5962223563213911, -297.4047404294462353, -287.6482577032830932 ) ) ;
#64541=CARTESIAN_POINT ( 'NONE',  ( -112.1219593623819293, -294.4544703416614766, -277.9730332437077891 ) ) ;
#64542=CARTESIAN_POINT ( 'NONE',  ( -46.12647284233057832, -298.5949075528844787, -193.9664810320958566 ) ) ;
#64543=CARTESIAN_POINT ( 'NONE',  ( -80.76975134200333173, -288.2288125048684719, -329.8331184021636204 ) ) ;
#64544=CARTESIAN_POINT ( 'NONE',  ( -62.73003454730126549, -275.7218535601055009, -199.7889342030195508 ) ) ;
#64545=CARTESIAN_POINT ( 'NONE',  ( -110.5408916181046663, -291.4464507817519916, -273.9323445476123311 ) ) ;
#64546=CARTESIAN_POINT ( 'NONE',  ( -113.0089288195105581, -273.2223907163500485, -256.1482573837037080 ) ) ;
#64548=CARTESIAN_POINT ( 'NONE',  ( -70.48093638989848841, -297.9360267548509569, -205.2789416701664322 ) ) ;
#64550=CARTESIAN_POINT ( 'NONE',  ( -98.11658978478460824, -281.1368372258975796, -225.7880170495248819 ) ) ;
#64551=CARTESIAN_POINT ( 'NONE',  ( 34.86783829909473553, -279.9142829084472623, -244.9227385442196123 ) ) ;
#64553=CARTESIAN_POINT ( 'NONE',  ( -61.20792641652438704, -282.7025496030915406, -343.5174562331770289 ) ) ;
#64554=CARTESIAN_POINT ( 'NONE',  ( 37.53755880876393292, -274.6808813665025468, -252.7992580946491614 ) ) ;
#64555=CARTESIAN_POINT ( 'NONE',  ( 23.96040918624438021, -279.3442538865699589, -225.1008505216792344 ) ) ;
#64556=CARTESIAN_POINT ( 'NONE',  ( -71.64682659988218916, -277.5998769855983710, -203.4649310619071514 ) ) ;
#64557=CARTESIAN_POINT ( 'NONE',  ( -110.1631684491267436, -271.2701662084614895, -259.4111670446782796 ) ) ;
#64558=CARTESIAN_POINT ( 'NONE',  ( 17.80331377923768343, -276.8412068593202662, -219.4533681940166048 ) ) ;
#64560=CARTESIAN_POINT ( 'NONE',  ( 12.21613416397512530, -290.7579585129442989, -213.5946854690895691 ) ) ;
#64561=CARTESIAN_POINT ( 'NONE',  ( -103.2158433414865613, -291.0736748591506284, -230.3885635273047967 ) ) ;
#64562=CARTESIAN_POINT ( 'NONE',  ( 22.91365519654061345, -278.1646343270953707, -315.2979690534764359 ) ) ;
#64563=CARTESIAN_POINT ( 'NONE',  ( -52.99431040300671469, -295.8510235791123932, -197.1299019693546200 ) ) ;
#64566=CARTESIAN_POINT ( 'NONE',  ( -101.0349512674058019, -283.0849446321930714, -230.6647968602192407 ) ) ;
#64568=CARTESIAN_POINT ( 'NONE',  ( -22.64620817748919990, -291.0393836648668753, -198.4502494022380290 ) ) ;
#64569=CARTESIAN_POINT ( 'NONE',  ( 34.26720205331995572, -285.9482259789573959, -290.1228118733554311 ) ) ;
#64572=CARTESIAN_POINT ( 'NONE',  ( -4.693292746754944567, -292.6219760205930811, -337.8962797370410271 ) ) ;
#64573=CARTESIAN_POINT ( 'NONE',  ( -66.33094126003810231, -281.9047330050557321, -340.9608113935905180 ) ) ;
#64574=CARTESIAN_POINT ( 'NONE',  ( -79.52868831286397722, -281.0716887577984835, -209.8078485298291014 ) ) ;
#64575=CARTESIAN_POINT ( 'NONE',  ( -110.5511282866018803, -286.0438813836186114, -247.6349951772083955 ) ) ;
#64576=CARTESIAN_POINT ( 'NONE',  ( -22.73866857007272557, -278.4762806424469090, -195.7373018772554474 ) ) ;
#64577=CARTESIAN_POINT ( 'NONE',  ( 25.69604982279730976, -288.0586454351242196, -307.2746640895851442 ) ) ;
#64578=CARTESIAN_POINT ( 'NONE',  ( -110.0716707475626208, -279.8306985265290336, -281.5738915562349689 ) ) ;
#64579=CARTESIAN_POINT ( 'NONE',  ( -109.6501033425589213, -279.2083592788199553, -281.5009811628668217 ) ) ;
#64580=CARTESIAN_POINT ( 'NONE',  ( -106.4284677089787152, -286.9255063519930218, -240.1402614045403254 ) ) ;
#64582=CARTESIAN_POINT ( 'NONE',  ( -36.53849372449802502, -297.8952692800526734, -193.3611399111292144 ) ) ;
#64583=CARTESIAN_POINT ( 'NONE',  ( 27.12911087680821609, -290.0382187882592575, -308.0846482415211653 ) ) ;
#64585=CARTESIAN_POINT ( 'NONE',  ( -88.47809603358389552, -286.1948066931273615, -334.5364918783848793 ) ) ;
#64587=CARTESIAN_POINT ( 'NONE',  ( -5.858382873068553209, -272.4649302057649720, -202.1055016194901270 ) ) ;
#64588=CARTESIAN_POINT ( 'NONE',  ( 36.99889954278052073, -292.1642111192376206, -287.1506240638425993 ) ) ;
#64589=CARTESIAN_POINT ( 'NONE',  ( -50.48842863854047636, -294.7322361177944572, -342.2301097032713528 ) ) ;
#64590=CARTESIAN_POINT ( 'NONE',  ( -35.93950333519057239, -287.5901792209469932, -196.6811234217904598 ) ) ;
#64591=CARTESIAN_POINT ( 'NONE',  ( 9.906434995802714027, -282.4730899709544474, -213.3242661542391261 ) ) ;
#64592=CARTESIAN_POINT ( 'NONE',  ( -5.852609018819689979, -290.0714752236990535, -339.9818292383837957 ) ) ;
#64593=CARTESIAN_POINT ( 'NONE',  ( 39.20929316504199136, -288.8819992766459563, -271.5269508892112071 ) ) ;
#64594=CARTESIAN_POINT ( 'NONE',  ( -56.81428319239153524, -285.3034222904404373, -342.7891453937122606 ) ) ;
#64595=CARTESIAN_POINT ( 'NONE',  ( -87.09357517439562457, -277.8893587537450571, -329.1995019790025481 ) ) ;
#64597=CARTESIAN_POINT ( 'NONE',  ( 36.37357847863370353, -291.8442372682825976, -287.0137689841113797 ) ) ;
#64598=CARTESIAN_POINT ( 'NONE',  ( 38.87096376473871118, -281.5228323519633591, -281.3442808633764116 ) ) ;
#64599=CARTESIAN_POINT ( 'NONE',  ( -92.04857262981425947, -275.1208828734801273, -220.1623814348911026 ) ) ;
#64600=CARTESIAN_POINT ( 'NONE',  ( -110.4542110544635705, -286.8376638359844719, -287.0812184334320705 ) ) ;
#64601=CARTESIAN_POINT ( 'NONE',  ( 33.23463610996259376, -274.1556528283517764, -298.6623260770533648 ) ) ;
#64602=CARTESIAN_POINT ( 'NONE',  ( -37.00175247351368313, -279.5641744234774251, -197.3003701252258111 ) ) ;
#64603=CARTESIAN_POINT ( 'NONE',  ( 32.66314985962230821, -277.1562290101872463, -301.4630422911588994 ) ) ;
#64604=CARTESIAN_POINT ( 'NONE',  ( -106.3647712631773032, -298.3167014589556061, -244.6956008299699192 ) ) ;
#64605=CARTESIAN_POINT ( 'NONE',  ( -94.23285773053657977, -282.9084798875504134, -321.9191117915657969 ) ) ;
#64606=CARTESIAN_POINT ( 'NONE',  ( -84.49158020638169830, -293.1526298000211455, -213.3097129208200613 ) ) ;
#64607=CARTESIAN_POINT ( 'NONE',  ( -113.3842125283154303, -274.2237454229970126, -264.7061221987347608 ) ) ;
#64608=CARTESIAN_POINT ( 'NONE',  ( -52.46463686376164759, -275.1776685771734492, -195.3097228702839629 ) ) ;
#64609=CARTESIAN_POINT ( 'NONE',  ( 21.14212687015213277, -296.1957981138944547, -317.0684954534502822 ) ) ;
#64610=CARTESIAN_POINT ( 'NONE',  ( -90.20703009310348364, -281.8011817663539205, -323.3988218308208502 ) ) ;
#64611=CARTESIAN_POINT ( 'NONE',  ( -113.6446014449358159, -290.3510891343242406, -259.7920564469905003 ) ) ;
#64612=CARTESIAN_POINT ( 'NONE',  ( -0.6839831367113394789, -274.5831523463790518, -335.4431223416971761 ) ) ;
#64613=CARTESIAN_POINT ( 'NONE',  ( -29.56505340102581059, -287.7492115842060230, -194.5589796193584107 ) ) ;
#64614=CARTESIAN_POINT ( 'NONE',  ( -110.4320055276906913, -289.3899588975598931, -276.6427679477179709 ) ) ;
#64616=CARTESIAN_POINT ( 'NONE',  ( -97.70537402949625516, -288.4964337440296163, -317.2101645927253912 ) ) ;
#64617=CARTESIAN_POINT ( 'NONE',  ( -85.93993655389900255, -291.0236200093633556, -215.7926150303602526 ) ) ;
#64619=CARTESIAN_POINT ( 'NONE',  ( 33.76093392611535648, -288.9997416855713368, -299.2412454452308452 ) ) ;
#64620=CARTESIAN_POINT ( 'NONE',  ( -92.73990890969220402, -278.2083216359442872, -317.9334413505611678 ) ) ;
#64621=CARTESIAN_POINT ( 'NONE',  ( 29.21422807408838551, -291.9754562643007034, -232.2586124192931436 ) ) ;
#64622=CARTESIAN_POINT ( 'NONE',  ( -113.0351415636737045, -285.0301188652370570, -284.2111747879503127 ) ) ;
#64623=CARTESIAN_POINT ( 'NONE',  ( -114.3196430519276134, -284.8901233486786282, -269.9861584539343653 ) ) ;
#64624=CARTESIAN_POINT ( 'NONE',  ( -30.26455934443297835, -280.4772882975129846, -197.6333683028722703 ) ) ;
#64625=CARTESIAN_POINT ( 'NONE',  ( -112.5841113068936181, -271.3072920273854152, -296.3762234298543490 ) ) ;
#64626=CARTESIAN_POINT ( 'NONE',  ( 159.9294595360192375, 220.4978701958970078, -204.6380096544159528 ) ) ;
#64627=CARTESIAN_POINT ( 'NONE',  ( -13.62517624662293514, -91.77141949113919850, -356.5202330857019319 ) ) ;
#64628=CARTESIAN_POINT ( 'NONE',  ( -108.0936030651267288, -271.9969844300305226, -251.5451928909460548 ) ) ;
#64629=CARTESIAN_POINT ( 'NONE',  ( -2.755730099628803664, -273.4411431380925706, -205.7233832493250532 ) ) ;
#64630=CARTESIAN_POINT ( 'NONE',  ( -11.08410929350230134, -294.2266883857589619, -342.7368343112370326 ) ) ;
#64631=CARTESIAN_POINT ( 'NONE',  ( 201.9261197471746527, 289.7920994275355042, -82.41291490543511600 ) ) ;
#64632=CARTESIAN_POINT ( 'NONE',  ( -24.22755737512878227, -272.9009294774529053, -194.9327814821474760 ) ) ;
#64633=CARTESIAN_POINT ( 'NONE',  ( -41.96860252685179660, -299.8536385514914855, -196.2702463755994131 ) ) ;
#64634=CARTESIAN_POINT ( 'NONE',  ( -37.25070687912403145, -290.3661654521764603, -343.8542142568012423 ) ) ;
#64635=CARTESIAN_POINT ( 'NONE',  ( -110.0084034461427649, -291.7639882115923911, -260.3002605963773703 ) ) ;
#64637=CARTESIAN_POINT ( 'NONE',  ( -89.45738539644557363, -298.2808080211027573, -213.9262081998626286 ) ) ;
#64638=CARTESIAN_POINT ( 'NONE',  ( -33.24146853771588894, -286.5973812609461788, -197.3648607540476405 ) ) ;
#64639=CARTESIAN_POINT ( 'NONE',  ( 38.16465939731381951, -294.1764408385868705, -256.1151188210793634 ) ) ;
#64640=CARTESIAN_POINT ( 'NONE',  ( 0.5156907188606600911, -295.0539999411656140, -337.3564686226543472 ) ) ;
#64641=CARTESIAN_POINT ( 'NONE',  ( 33.44658187695048923, -293.9541882321916546, -288.1942090019722400 ) ) ;
#64642=VERTEX_POINT ( 'NONE', #39291 ) ;
#64643=CARTESIAN_POINT ( 'NONE',  ( -35.58229619559588741, -275.9941843413375864, -194.8087156026683147 ) ) ;
#64645=CARTESIAN_POINT ( 'NONE',  ( -113.9820002251451854, -278.1517710701338615, -263.0135606456025812 ) ) ;
#64646=CARTESIAN_POINT ( 'NONE',  ( -29.88903592127486419, -272.5479225923768354, -196.9383816469575095 ) ) ;
#64647=CARTESIAN_POINT ( 'NONE',  ( -33.80335719823045793, -299.3024927178125267, -196.9632974387495494 ) ) ;
#64648=CARTESIAN_POINT ( 'NONE',  ( 31.33482123755863213, -276.1553232386330592, -244.9260268507880483 ) ) ;
#64649=CARTESIAN_POINT ( 'NONE',  ( -55.11858395926975618, -275.5867060649601967, -196.4831347091606801 ) ) ;
#64650=CARTESIAN_POINT ( 'NONE',  ( 13.74908610780818563, -274.3608453319600358, -325.8228932254388042 ) ) ;
#64651=CARTESIAN_POINT ( 'NONE',  ( -52.66453942647950015, -298.5021706263122496, -198.8311675679265420 ) ) ;
#64652=CARTESIAN_POINT ( 'NONE',  ( -7.768034845374670816, -293.2315518164654122, -337.7600629323433168 ) ) ;
#64654=CARTESIAN_POINT ( 'NONE',  ( -112.3431469562897718, -279.2592208192483554, -253.2056559578821293 ) ) ;
#64656=CARTESIAN_POINT ( 'NONE',  ( -24.32751793415375730, -277.0481772360093373, -342.2431409196510685 ) ) ;
#64657=CARTESIAN_POINT ( 'NONE',  ( -49.25133195738426650, -284.5883691534731952, -194.7335325952351184 ) ) ;
#64658=CARTESIAN_POINT ( 'NONE',  ( -62.26183845851925724, -299.7289374515877967, -199.4455686927227021 ) ) ;
#64659=CARTESIAN_POINT ( 'NONE',  ( 82.61792974232589870, -301.9867274997020559, -195.9612250618527582 ) ) ;
#64660=CARTESIAN_POINT ( 'NONE',  ( 16.09939010480643518, -286.0319170857039808, -220.3761228436786155 ) ) ;
#64661=CARTESIAN_POINT ( 'NONE',  ( -95.57442760217497835, -277.4275409691693994, -224.6578702495095854 ) ) ;
#64662=CARTESIAN_POINT ( 'NONE',  ( -87.92255680118810801, -277.9031965931899322, -216.8402512598194392 ) ) ;
#64663=CARTESIAN_POINT ( 'NONE',  ( -108.3908751323648687, -286.2398479179511241, -294.5401914223550079 ) ) ;
#64664=CARTESIAN_POINT ( 'NONE',  ( -29.65667141302510146, -278.1579032777492557, -343.4059370589894797 ) ) ;
#64666=CARTESIAN_POINT ( 'NONE',  ( 25.49651181853103310, -273.3769838959071876, -227.2357833895700310 ) ) ;
#64667=CARTESIAN_POINT ( 'NONE',  ( -8.938874093622489525, -275.0850226053447614, -202.9486001580102936 ) ) ;
#64668=CARTESIAN_POINT ( 'NONE',  ( 18.74336585502158314, -282.8570347907921132, -220.2968544067906578 ) ) ;
#64670=CARTESIAN_POINT ( 'NONE',  ( 37.13330947979401486, -289.3087279003423760, -257.5263366218349006 ) ) ;
#64671=CARTESIAN_POINT ( 'NONE',  ( -7.618056273180739524, -290.4415798260847055, -201.4888150816176449 ) ) ;
#64673=CARTESIAN_POINT ( 'NONE',  ( -43.50690766080450800, -272.6576082382700292, -197.0759630084056653 ) ) ;
#64674=CARTESIAN_POINT ( 'NONE',  ( 35.43199096186359043, -291.5015898185102969, -255.7031724204378236 ) ) ;
#64675=CARTESIAN_POINT ( 'NONE',  ( 142.9247625494386114, 180.1091408837567371, -243.7470944784683127 ) ) ;
#64677=CARTESIAN_POINT ( 'NONE',  ( -51.57512821632436584, -287.7109146105174773, -345.3285594210822183 ) ) ;
#64678=CARTESIAN_POINT ( 'NONE',  ( -89.44481840427226871, -285.4008904394593173, -322.6985455075389950 ) ) ;
#64679=CARTESIAN_POINT ( 'NONE',  ( -15.68057846130173338, -284.5683803552137761, -197.4725982742139081 ) ) ;
#64680=CARTESIAN_POINT ( 'NONE',  ( 3.734043674811053926, -283.9130063366745844, -331.4814122082969448 ) ) ;
#64681=CARTESIAN_POINT ( 'NONE',  ( -84.95915126408831952, -284.5320359941491120, -325.9055153037097625 ) ) ;
#64682=CARTESIAN_POINT ( 'NONE',  ( -110.7214783712935287, -292.7510963614427055, -253.2200867269018829 ) ) ;
#64683=CARTESIAN_POINT ( 'NONE',  ( -3.839146081167362112, -274.8153525920508287, -201.0406029347051913 ) ) ;
#64684=CARTESIAN_POINT ( 'NONE',  ( -112.8141733872998458, -288.5856577071867264, -273.9970464185900028 ) ) ;
#64685=CARTESIAN_POINT ( 'NONE',  ( -9.211819363219134971, -276.6943583624274083, -342.0389374817232806 ) ) ;
#64686=CARTESIAN_POINT ( 'NONE',  ( 2.467899391831208433, -296.4960477200129958, -333.5653794872768572 ) ) ;
#64688=CARTESIAN_POINT ( 'NONE',  ( -54.49178911615187815, -300.3376638359845856, -195.3683826091709363 ) ) ;
#64689=CARTESIAN_POINT ( 'NONE',  ( -92.94312924394861852, -282.5566499234737421, -318.4398684498609668 ) ) ;
#64690=CARTESIAN_POINT ( 'NONE',  ( -8.287617366962106047, -278.4323822918511269, -201.2034140387603713 ) ) ;
#64691=CARTESIAN_POINT ( 'NONE',  ( -15.08038611036102772, -296.7263302168457244, -194.1670541500574529 ) ) ;
#64692=CARTESIAN_POINT ( 'NONE',  ( 35.20618119564122850, -275.0243867483887925, -279.7476395292657116 ) ) ;
#64693=CARTESIAN_POINT ( 'NONE',  ( -33.49138783198756641, -293.6215868464246341, -196.7558249745424916 ) ) ;
#64694=CARTESIAN_POINT ( 'NONE',  ( 33.87376742875545688, -294.2681414203026407, -253.2264326632809741 ) ) ;
#64695=CARTESIAN_POINT ( 'NONE',  ( -5.984411523326589766, -295.9636969250614698, -340.1466374372848236 ) ) ;
#64696=CARTESIAN_POINT ( 'NONE',  ( -104.7613973143008508, -296.7608554442849709, -242.3685397553790040 ) ) ;
#64697=CARTESIAN_POINT ( 'NONE',  ( -110.2899331885888472, -292.3285804382922493, -287.7839749952365196 ) ) ;
#64698=CARTESIAN_POINT ( 'NONE',  ( -61.22965565113217679, -283.5205110774961668, -343.6176596128119058 ) ) ;
#64699=CARTESIAN_POINT ( 'NONE',  ( 15.18797384254098048, -272.9239223906698726, -215.7631433736737279 ) ) ;
#64700=CARTESIAN_POINT ( 'NONE',  ( -7.341170417150187255, -286.2680397477288921, -199.3892431055238035 ) ) ;
#64701=CARTESIAN_POINT ( 'NONE',  ( -15.88446999061008214, -278.7532821440228190, -341.9096210679908268 ) ) ;
#64702=CARTESIAN_POINT ( 'NONE',  ( -52.12475683126957904, -284.9169705440760367, -198.6333710369109724 ) ) ;
#64703=CARTESIAN_POINT ( 'NONE',  ( -2.746512316524156283, -286.5945727672310568, -336.9056416640585780 ) ) ;
#64704=CARTESIAN_POINT ( 'NONE',  ( -82.08396892746139883, -205.6231916066184624, -355.0661004095303497 ) ) ;
#64705=CARTESIAN_POINT ( 'NONE',  ( -42.67236761581845883, -285.4907690970902649, -197.4816688080940708 ) ) ;
#64706=CARTESIAN_POINT ( 'NONE',  ( 38.88462032965388460, -282.8590533884334945, -278.4612095447548086 ) ) ;
#64707=CARTESIAN_POINT ( 'NONE',  ( -87.24061519651937147, -288.7863501311317691, -328.7654861955888350 ) ) ;
#64708=CARTESIAN_POINT ( 'NONE',  ( -104.1025956989616645, -280.6330467546099499, -233.6266214402496644 ) ) ;
#64709=CARTESIAN_POINT ( 'NONE',  ( -111.6112618883273342, -280.0991799311533441, -251.9407611819490285 ) ) ;
#64710=CARTESIAN_POINT ( 'NONE',  ( -16.91968232517835347, -280.1566730169467405, -200.2758756462107783 ) ) ;
#64711=CARTESIAN_POINT ( 'NONE',  ( -82.07645398955150995, -275.4191489984258396, -210.5413387400024021 ) ) ;
#64712=CARTESIAN_POINT ( 'NONE',  ( 37.78392580287127345, -293.7640804251029181, -287.3067295327173838 ) ) ;
#64713=CARTESIAN_POINT ( 'NONE',  ( -45.56820836405109532, -287.1770306973840547, -344.5512208532886689 ) ) ;
#64714=CARTESIAN_POINT ( 'NONE',  ( -30.78661262731542436, -293.7336892799484644, -194.3913786101214782 ) ) ;
#64715=CARTESIAN_POINT ( 'NONE',  ( -101.4783850978630682, -295.9557233611561173, -234.8546155652680909 ) ) ;
#64716=CARTESIAN_POINT ( 'NONE',  ( 28.13301183152943707, -283.9461790962319014, -305.7782930399445149 ) ) ;
#64717=CARTESIAN_POINT ( 'NONE',  ( -104.9830836151757012, -295.8504864989470207, -297.8698570785538209 ) ) ;
#64719=CARTESIAN_POINT ( 'NONE',  ( 15.21627682194673881, -293.8528386752993242, -214.4388500009942220 ) ) ;
#64720=CARTESIAN_POINT ( 'NONE',  ( -11.71517612459890323, -281.0461312422029323, -201.8446504206062002 ) ) ;
#64721=CARTESIAN_POINT ( 'NONE',  ( -5.201826432360350694, -273.5236673502162148, -200.6485026771076718 ) ) ;
#64722=CARTESIAN_POINT ( 'NONE',  ( -87.31189124135524082, -290.3787590148033928, -328.8801131787508325 ) ) ;
#64723=CARTESIAN_POINT ( 'NONE',  ( -80.87157440323589697, -281.7752299061435224, -332.4366935245436139 ) ) ;
#64724=CARTESIAN_POINT ( 'NONE',  ( -110.7603945291620704, -290.5925957306848204, -293.6747970450525145 ) ) ;
#64725=CARTESIAN_POINT ( 'NONE',  ( 34.03224866874087695, -288.0895464783077955, -285.8420643823129126 ) ) ;
#64727=CARTESIAN_POINT ( 'NONE',  ( -40.95418676001914093, -138.9741238729967563, -362.5036135750506219 ) ) ;
#64728=CARTESIAN_POINT ( 'NONE',  ( -30.40625769401537326, -125.0523020468976227, -360.4922289175208903 ) ) ;
#64729=CARTESIAN_POINT ( 'NONE',  ( -110.4683760289727132, -275.8380690714489560, -287.0191576251351080 ) ) ;
#64730=CARTESIAN_POINT ( 'NONE',  ( -108.4441905920833449, -277.9762095854501354, -253.1263398486288168 ) ) ;
#64732=CARTESIAN_POINT ( 'NONE',  ( -30.21872262107783058, -279.0645635344039306, -197.3483040412711205 ) ) ;
#64733=CARTESIAN_POINT ( 'NONE',  ( 37.92561291005537782, -275.0161551272126985, -254.1564242120706183 ) ) ;
#64734=CARTESIAN_POINT ( 'NONE',  ( 190.6894252310336526, 268.2488200997306649, -138.1386062953752401 ) ) ;
#64735=CARTESIAN_POINT ( 'NONE',  ( -28.27675326729536920, -278.7396257917655475, -194.4367416818954553 ) ) ;
#64736=CARTESIAN_POINT ( 'NONE',  ( -105.6279316232924117, -282.1755075324275595, -300.5080479741156410 ) ) ;
#64737=CARTESIAN_POINT ( 'NONE',  ( -106.8552173197297464, -298.7105353221991777, -239.5414464643715746 ) ) ;
#64738=CARTESIAN_POINT ( 'NONE',  ( -17.42183542464008639, -292.8084383920509026, -200.0149024682672518 ) ) ;
#64740=CARTESIAN_POINT ( 'NONE',  ( -61.43236756502461304, -288.0565608071930797, -339.7936983753351683 ) ) ;
#64741=CARTESIAN_POINT ( 'NONE',  ( -49.71103001416717149, -274.5499064965100615, -194.4106607895813283 ) ) ;
#64742=CARTESIAN_POINT ( 'NONE',  ( -96.28137092940995956, -273.1562831760284666, -227.2060860369406043 ) ) ;
#64746=CARTESIAN_POINT ( 'NONE',  ( -66.82358179535859222, -281.5890009728792052, -200.7900546510638264 ) ) ;
#64749=CARTESIAN_POINT ( 'NONE',  ( 32.26578842316664009, -282.3258787783213393, -247.2007033208231235 ) ) ;
#64750=CARTESIAN_POINT ( 'NONE',  ( -14.55330129389469107, -282.1035608530683021, -197.8169053525276411 ) ) ;
#64751=CARTESIAN_POINT ( 'NONE',  ( -110.2273431385451090, -283.7114544507192591, -262.7136045495970507 ) ) ;
#64753=CARTESIAN_POINT ( 'NONE',  ( -111.3924216447653350, -280.4804229353496225, -265.1308100496698898 ) ) ;
#64754=CARTESIAN_POINT ( 'NONE',  ( 23.02274142192727524, -274.6170503720201737, -312.7197485551346290 ) ) ;
#64757=CARTESIAN_POINT ( 'NONE',  ( -82.44322468574870300, -278.4536609344096405, -332.5705328858309144 ) ) ;
#64758=VERTEX_POINT ( 'NONE', #90413 ) ;
#64759=CARTESIAN_POINT ( 'NONE',  ( -96.60896541417068306, -276.4745423961463189, -318.6102098068657824 ) ) ;
#64762=CARTESIAN_POINT ( 'NONE',  ( -85.04132537923237578, -285.6866718536684857, -328.6976635664029232 ) ) ;
#64763=CARTESIAN_POINT ( 'NONE',  ( 35.36620734229189367, -292.8622300481466141, -278.9396012712676907 ) ) ;
#64765=CARTESIAN_POINT ( 'NONE',  ( 31.59236124351189900, -287.3406237297907069, -304.5606190968654232 ) ) ;
#64766=CARTESIAN_POINT ( 'NONE',  ( -60.27157930858084001, -283.9905997117509742, -199.9892865950615999 ) ) ;
#64767=CARTESIAN_POINT ( 'NONE',  ( -72.64083230934006963, -284.1498186324519111, -205.7763137370687616 ) ) ;
#64768=CARTESIAN_POINT ( 'NONE',  ( 18.57659422719453701, -286.4742968597512913, -318.9261553990029938 ) ) ;
#64769=CARTESIAN_POINT ( 'NONE',  ( 35.96326199687488412, -282.8054648719526085, -274.0371255526139294 ) ) ;
#64770=CARTESIAN_POINT ( 'NONE',  ( 22.06469534346717865, -272.9245274711426532, -224.5594142714235204 ) ) ;
#64771=CARTESIAN_POINT ( 'NONE',  ( -91.32175294512047969, -283.6995970974033412, -216.5782739480239343 ) ) ;
#64772=CARTESIAN_POINT ( 'NONE',  ( -55.55917935315227396, -297.2867801693913634, -343.1149776490763088 ) ) ;
#64773=CARTESIAN_POINT ( 'NONE',  ( -5.526215443668818672, -284.4695189624267755, -202.2596982827882073 ) ) ;
#64774=CARTESIAN_POINT ( 'NONE',  ( -109.2721266827422113, -279.3115620963374113, -284.1903962125614953 ) ) ;
#64775=CARTESIAN_POINT ( 'NONE',  ( 32.15443894610123721, -289.1778863349051107, -241.5841114757561172 ) ) ;
#64778=CARTESIAN_POINT ( 'NONE',  ( 22.89607022198499209, -296.0915531886318490, -315.9760850922224904 ) ) ;
#64779=CARTESIAN_POINT ( 'NONE',  ( -112.1518307317253687, -276.6204681987582035, -265.0277320497596634 ) ) ;
#64780=CARTESIAN_POINT ( 'NONE',  ( -111.0743301631594164, -290.0211409249805570, -248.7357142002668411 ) ) ;
#64781=CARTESIAN_POINT ( 'NONE',  ( 18.56528400437992588, -292.6309045405507732, -318.5555759000557714 ) ) ;
#64782=CARTESIAN_POINT ( 'NONE',  ( -9.042077963082315151, -279.1150146316199425, -202.5350546731747556 ) ) ;
#64783=CARTESIAN_POINT ( 'NONE',  ( -92.16686870826306688, -271.3409231206380241, -219.9883575876487782 ) ) ;
#64784=CARTESIAN_POINT ( 'NONE',  ( 0.1462936821208547233, -293.8778019906856116, -207.1480354904180956 ) ) ;
#64785=CARTESIAN_POINT ( 'NONE',  ( 21.31550574532285580, -278.6948066931273615, -317.0979686699210447 ) ) ;
#64786=CARTESIAN_POINT ( 'NONE',  ( -71.77861896020590393, -293.9788779815642670, -338.4552174061741425 ) ) ;
#64787=CARTESIAN_POINT ( 'NONE',  ( -29.06337183588486539, -290.5456214251294114, -343.6953507472241540 ) ) ;
#64788=CARTESIAN_POINT ( 'NONE',  ( -58.63299134959753900, -290.0203647536698668, -197.4182983922744086 ) ) ;
#64789=CARTESIAN_POINT ( 'NONE',  ( -72.62555981011973927, -290.9543782178983520, -334.9399393092668902 ) ) ;
#64791=CARTESIAN_POINT ( 'NONE',  ( -56.09714401786292370, -290.1026763328785023, -341.1303718904458719 ) ) ;
#64794=CARTESIAN_POINT ( 'NONE',  ( -113.7925274205179420, -291.8178809281456552, -265.5362113576314869 ) ) ;
#64795=CARTESIAN_POINT ( 'NONE',  ( 19.83491766168293680, -278.8951409268548787, -221.2574672631898807 ) ) ;
#64796=CARTESIAN_POINT ( 'NONE',  ( -95.11439130822638788, -291.1804236143703974, -225.7369524015254569 ) ) ;
#64797=CARTESIAN_POINT ( 'NONE',  ( -96.80381148168737582, -279.5424952283311768, -221.4529764343397744 ) ) ;
#64798=CARTESIAN_POINT ( 'NONE',  ( 2.079664409559733418, -282.2061615606692158, -336.4799527386016393 ) ) ;
#64799=CARTESIAN_POINT ( 'NONE',  ( 19.30299774851949834, -284.8699592232133000, -221.2044413910540470 ) ) ;
#64801=CARTESIAN_POINT ( 'NONE',  ( 35.69654490444180084, -279.8648885396994501, -283.7092805312842643 ) ) ;
#64802=CARTESIAN_POINT ( 'NONE',  ( -112.3553692517585318, -282.5211962451222121, -272.7591947047818053 ) ) ;
#64804=CARTESIAN_POINT ( 'NONE',  ( -111.1616768445554158, -276.7874002616387088, -289.7339702682834854 ) ) ;
#64805=CARTESIAN_POINT ( 'NONE',  ( -112.6919010022137684, -283.6551827870788998, -255.8078313250566964 ) ) ;
#64806=CARTESIAN_POINT ( 'NONE',  ( -100.8630312116333130, -273.8524736366951515, -233.9598768378228328 ) ) ;
#64808=CARTESIAN_POINT ( 'NONE',  ( -104.2905159907218433, -292.5668962447462604, -239.3079946676770646 ) ) ;
#64809=CARTESIAN_POINT ( 'NONE',  ( -27.09365417432926293, -275.6051259247636267, -194.5876656206886821 ) ) ;
#64810=CARTESIAN_POINT ( 'NONE',  ( -5.060556969323847021, -276.2818449749674983, -335.8732203546749133 ) ) ;
#64811=CARTESIAN_POINT ( 'NONE',  ( 19.50454607328424572, -296.2306114705191931, -319.3041680958199322 ) ) ;
#64812=CARTESIAN_POINT ( 'NONE',  ( -36.08471351486991807, -289.2035130133343159, -347.3639678062371559 ) ) ;
#64813=CARTESIAN_POINT ( 'NONE',  ( -6.789770406774897182, -278.5298736902030328, -201.2392684336859645 ) ) ;
#64814=CARTESIAN_POINT ( 'NONE',  ( -73.43183545768000897, -291.4202271591936437, -202.3278228347040226 ) ) ;
#64815=CARTESIAN_POINT ( 'NONE',  ( -47.01371349523969911, -290.9850267683520997, -197.7673124260751081 ) ) ;
#64816=CARTESIAN_POINT ( 'NONE',  ( -28.02228166383421382, -292.9338161723024996, -344.8317667229835024 ) ) ;
#64819=CARTESIAN_POINT ( 'NONE',  ( 12.95005438590779079, -292.2853845396969632, -217.3636853140565393 ) ) ;
#64821=CARTESIAN_POINT ( 'NONE',  ( 27.33386217378598815, -279.4809262143061233, -301.5434626090942629 ) ) ;
#64822=CARTESIAN_POINT ( 'NONE',  ( -111.3683060265434790, -295.3555966267059603, -290.6806118878683378 ) ) ;
#64823=CARTESIAN_POINT ( 'NONE',  ( -112.5168896377793715, -286.0496396853866941, -255.8728551344655671 ) ) ;
#64824=CARTESIAN_POINT ( 'NONE',  ( 35.65515926231452681, -287.3944036716816868, -271.0382617056125127 ) ) ;
#64825=CARTESIAN_POINT ( 'NONE',  ( 35.30591346791839413, -276.9096467825079344, -257.9156701971692769 ) ) ;
#64826=CARTESIAN_POINT ( 'NONE',  ( 29.86471317700003070, -292.0035824842242391, -302.9632282876810336 ) ) ;
#64827=CARTESIAN_POINT ( 'NONE',  ( 36.63343835856003494, -295.2813660653665124, -267.9835358271650989 ) ) ;
#64828=CARTESIAN_POINT ( 'NONE',  ( 16.81382174454465073, -275.0541120063930407, -319.9208516148004833 ) ) ;
#64831=CARTESIAN_POINT ( 'NONE',  ( -98.26032971053273002, -295.5905422204444335, -317.4213438791338717 ) ) ;
#64832=CARTESIAN_POINT ( 'NONE',  ( 23.14579132524312044, -290.0670783776265012, -313.7497982710228825 ) ) ;
#64833=CARTESIAN_POINT ( 'NONE',  ( 201.4659665719736097, 295.2841405640494372, -54.00000000003616663 ) ) ;
#64834=CARTESIAN_POINT ( 'NONE',  ( -46.10824021721057875, -299.0230967147259094, -194.1729280565668034 ) ) ;
#64835=CARTESIAN_POINT ( 'NONE',  ( 13.20405196619358534, -287.4326782644043305, -217.4801194004139120 ) ) ;
#64837=CARTESIAN_POINT ( 'NONE',  ( -92.89516848816764139, -278.3381443315037700, -217.3075237313009609 ) ) ;
#64838=CARTESIAN_POINT ( 'NONE',  ( 34.35944555851182969, -294.5560902270212864, -298.1506572658657319 ) ) ;
#64839=CARTESIAN_POINT ( 'NONE',  ( -72.62008019093364908, -287.6536990479655174, -337.4259295986626057 ) ) ;
#64840=CARTESIAN_POINT ( 'NONE',  ( -64.25481809761065222, -295.7271921037819880, -342.4820467942532218 ) ) ;
#64841=CARTESIAN_POINT ( 'NONE',  ( 29.51111778551385356, -294.2804839683433897, -299.7343749299255364 ) ) ;
#64845=CARTESIAN_POINT ( 'NONE',  ( -3.811636168764664045, -288.0065628828402851, -201.8015367330476693 ) ) ;
#64846=CARTESIAN_POINT ( 'NONE',  ( 44.71564893372296723, -285.0523547857347353, -270.3937649182068412 ) ) ;
#64847=CARTESIAN_POINT ( 'NONE',  ( -101.8012386096887809, -278.4532664994625861, -228.3329224186558406 ) ) ;
#64848=CARTESIAN_POINT ( 'NONE',  ( -6.474565824664024305, -284.6460189540223382, -338.5459087240757867 ) ) ;
#64849=CARTESIAN_POINT ( 'NONE',  ( -109.6728099937270144, -282.8141203514168751, -294.9947705315508983 ) ) ;
#64850=CARTESIAN_POINT ( 'NONE',  ( 6.676831608318957834, -286.5286358453101343, -330.4560264799730476 ) ) ;
#64851=CARTESIAN_POINT ( 'NONE',  ( 38.47165267407766009, -277.4224054792246648, -271.1349953099904724 ) ) ;
#64852=CARTESIAN_POINT ( 'NONE',  ( -43.48813426490022493, -274.3057975246948104, -197.5483911267091912 ) ) ;
#64854=CARTESIAN_POINT ( 'NONE',  ( -68.74315866602611891, -294.1585618424003314, -336.8218534164845437 ) ) ;
#64855=CARTESIAN_POINT ( 'NONE',  ( -99.17509273922071600, -278.0151929862021234, -309.2580087107771760 ) ) ;
#64856=CARTESIAN_POINT ( 'NONE',  ( -59.75701063985993500, -279.1026896116431431, -200.7272368739066337 ) ) ;
#64857=CARTESIAN_POINT ( 'NONE',  ( -38.36712413510893782, -275.1192458227329212, -193.6770843333568166 ) ) ;
#64858=CARTESIAN_POINT ( 'NONE',  ( -113.8363169450933015, -277.2958864952799445, -274.4332569294710993 ) ) ;
#64859=CARTESIAN_POINT ( 'NONE',  ( -78.81524805502048991, -207.3136162032604659, -354.6738105741294476 ) ) ;
#64860=CARTESIAN_POINT ( 'NONE',  ( -99.45325900190022139, -298.5717068622785177, -225.8553818588908371 ) ) ;
#64862=CARTESIAN_POINT ( 'NONE',  ( -106.6662871844225293, -275.4805209788417528, -237.0123917617630980 ) ) ;
#64864=AXIS2_PLACEMENT_3D ( 'NONE', #8069, #36958, #65871 ) ;
#64866=CARTESIAN_POINT ( 'NONE',  ( -99.88016898236796237, -286.1578177189136341, -232.0130187540122790 ) ) ;
#64867=CARTESIAN_POINT ( 'NONE',  ( -54.75445595234098306, -287.5914494448043115, -196.3964646278142254 ) ) ;
#64868=CARTESIAN_POINT ( 'NONE',  ( 35.78256163974624826, -286.8738185703300019, -268.3178757458759947 ) ) ;
#64869=CARTESIAN_POINT ( 'NONE',  ( -112.4663634463238537, -283.8519408983603398, -286.9687025415564108 ) ) ;
#64870=CARTESIAN_POINT ( 'NONE',  ( -5.191769931830755525, -278.8824211001969502, -203.9320399657017902 ) ) ;
#64871=CARTESIAN_POINT ( 'NONE',  ( -68.08042643044159092, -287.5045852517947651, -202.7889625602731201 ) ) ;
#64872=CARTESIAN_POINT ( 'NONE',  ( 7.580146836008246680, -279.1573380924104413, -211.8779183624485256 ) ) ;
#64873=CARTESIAN_POINT ( 'NONE',  ( -81.09967080430737951, -278.9760764028137032, -329.4075698570590589 ) ) ;
#64874=CARTESIAN_POINT ( 'NONE',  ( 26.68743840101996057, -275.5629732485845693, -235.0668034416792977 ) ) ;
#64875=CARTESIAN_POINT ( 'NONE',  ( -75.47937926186932600, -288.3440620631050706, -336.7954927367333653 ) ) ;
#64876=CARTESIAN_POINT ( 'NONE',  ( -41.55004729521917284, -283.9065770576856380, -347.1365299970082674 ) ) ;
#64877=CARTESIAN_POINT ( 'NONE',  ( 9.176584106296594712, -282.9246678125839480, -331.6438735908672584 ) ) ;
#64881=CARTESIAN_POINT ( 'NONE',  ( -26.30077655663473735, -290.7734659646230853, -345.3171283168143191 ) ) ;
#64882=CARTESIAN_POINT ( 'NONE',  ( -112.8758573263596077, -289.0839120606259485, -282.5220953043358350 ) ) ;
#64883=CARTESIAN_POINT ( 'NONE',  ( -94.78984615908625244, -272.2498265784545310, -224.9395485849079250 ) ) ;
#64885=CARTESIAN_POINT ( 'NONE',  ( 32.13436253922301944, -293.3250986967233302, -303.4456419533718190 ) ) ;
#64886=CARTESIAN_POINT ( 'NONE',  ( -75.08750103998879410, -288.0447196432907617, -333.6686178426868992 ) ) ;
#64887=CARTESIAN_POINT ( 'NONE',  ( 28.39671628957148997, -291.3359022868795591, -236.3547271435378150 ) ) ;
#64888=CARTESIAN_POINT ( 'NONE',  ( 35.84913324137321666, -288.8377696663205256, -276.4993495235758587 ) ) ;
#64889=CARTESIAN_POINT ( 'NONE',  ( 31.95455697924148097, -295.6233781216988632, -236.9535640164627637 ) ) ;
#64890=CARTESIAN_POINT ( 'NONE',  ( -26.41023446725840174, -290.9131880085710122, -344.5601995478144772 ) ) ;
#64891=CARTESIAN_POINT ( 'NONE',  ( -73.76761629400313325, -289.5694842315243704, -204.6102163961794815 ) ) ;
#64892=CARTESIAN_POINT ( 'NONE',  ( -5.161021176193295368, -294.4758340443110569, -202.6020382514811615 ) ) ;
#64893=CARTESIAN_POINT ( 'NONE',  ( -105.7890882556549172, -285.8400331174468647, -244.3157055993873712 ) ) ;
#64894=CARTESIAN_POINT ( 'NONE',  ( 27.87211595891487903, -295.0547921746466500, -232.9821584515795507 ) ) ;
#64897=CARTESIAN_POINT ( 'NONE',  ( -112.6978367782134711, -274.5675873361152526, -267.5800565663478778 ) ) ;
#64898=CARTESIAN_POINT ( 'NONE',  ( 35.51415487905948964, -280.6543400406660567, -263.1455633865182904 ) ) ;
#64899=CARTESIAN_POINT ( 'NONE',  ( -67.38345437760226275, -281.4459563558073683, -339.0954654058396613 ) ) ;
#64900=CARTESIAN_POINT ( 'NONE',  ( -108.7347667244529390, -296.1120958670094865, -241.8071133479353989 ) ) ;
#64901=CARTESIAN_POINT ( 'NONE',  ( 33.03221910872545664, -273.4900587956998379, -247.2726227099493883 ) ) ;
#64902=CARTESIAN_POINT ( 'NONE',  ( -108.5986083724690729, -276.9116082142066944, -248.8258625606869714 ) ) ;
#64903=CARTESIAN_POINT ( 'NONE',  ( -105.2240762792772557, -298.2424709397903371, -242.1968412317631021 ) ) ;
#64904=CARTESIAN_POINT ( 'NONE',  ( 35.48831257374818904, -294.8394577455441095, -259.8176760795727205 ) ) ;
#64906=CARTESIAN_POINT ( 'NONE',  ( 3.915857296505884211, -295.2833938693804043, -330.7797879609530582 ) ) ;
#64908=CARTESIAN_POINT ( 'NONE',  ( 36.49155210934362259, -285.7648286151041361, -285.4295508892598718 ) ) ;
#64909=CARTESIAN_POINT ( 'NONE',  ( -88.50184912708041907, -295.7937764394198439, -322.5055587534849337 ) ) ;
#64910=CARTESIAN_POINT ( 'NONE',  ( -88.32153722872978108, -283.7429556742942509, -328.1389503967723726 ) ) ;
#64911=CARTESIAN_POINT ( 'NONE',  ( 19.60574515177151511, -287.9231784482374792, -322.1758544495715455 ) ) ;
#64912=CARTESIAN_POINT ( 'NONE',  ( -91.49703810126871417, -297.7984831134086789, -322.7596501309698738 ) ) ;
#64913=CARTESIAN_POINT ( 'NONE',  ( 19.89487193438722556, -290.8839165013578167, -222.1532011199816452 ) ) ;
#64914=CARTESIAN_POINT ( 'NONE',  ( -109.4510998821137520, -278.0871982139832426, -243.6671527312089722 ) ) ;
#64915=CARTESIAN_POINT ( 'NONE',  ( -106.6379572354042153, -282.4809262143061233, -236.9535640164627068 ) ) ;
#64917=CARTESIAN_POINT ( 'NONE',  ( 36.02619794885956139, -286.3921050236789370, -273.7936192847289476 ) ) ;
#64920=CARTESIAN_POINT ( 'NONE',  ( -108.3672566232775978, -297.8901709505469171, -290.4063353878182738 ) ) ;
#64921=CARTESIAN_POINT ( 'NONE',  ( 24.10700271430414432, -282.3691655434998893, -224.9445657891542680 ) ) ;
#64922=CARTESIAN_POINT ( 'NONE',  ( -106.8674499587810516, -294.1930234440782783, -299.5578819612953794 ) ) ;
#64923=CARTESIAN_POINT ( 'NONE',  ( 34.72374258919094814, -281.3741612913639756, -282.1364928288355713 ) ) ;
#64924=CARTESIAN_POINT ( 'NONE',  ( -94.65015683057279716, -296.0208832418985025, -321.8078052166281395 ) ) ;
#64925=CARTESIAN_POINT ( 'NONE',  ( -96.66990747832352326, -298.6793800730595194, -226.6262897259971680 ) ) ;
#64926=CARTESIAN_POINT ( 'NONE',  ( 34.48791835814993334, -285.3294554416447113, -246.7453767825517730 ) ) ;
#64927=CARTESIAN_POINT ( 'NONE',  ( -111.0941241552230139, -280.3764921216308608, -284.0543474257601702 ) ) ;
#64929=CARTESIAN_POINT ( 'NONE',  ( -108.4003396995335180, -295.8446261396671275, -252.5875608071127090 ) ) ;
#64930=VERTEX_POINT ( 'NONE', #4270 ) ;
#64932=CARTESIAN_POINT ( 'NONE',  ( -6.552508724816060948, -284.6257539362730995, -338.3742056111131546 ) ) ;
#64933=LINE ( 'NONE', #42633, #79192 ) ;
#64934=CARTESIAN_POINT ( 'NONE',  ( -114.2704648735229114, -288.0523547857346784, -270.3284710469133074 ) ) ;
#64935=CARTESIAN_POINT ( 'NONE',  ( -11.92925525884559335, -275.9269183552944469, -342.9315191208891065 ) ) ;
#64936=CARTESIAN_POINT ( 'NONE',  ( -3.634370182412778760, -292.3433983063298456, -205.6091611591530466 ) ) ;
#64937=CARTESIAN_POINT ( 'NONE',  ( 35.17112336764623848, -283.2448801671390015, -283.5695907963116156 ) ) ;
#64938=CARTESIAN_POINT ( 'NONE',  ( -5.917680616117033665, -278.2321655745086559, -337.1505696092807511 ) ) ;
#64939=CARTESIAN_POINT ( 'NONE',  ( -41.50483637870826215, -284.7037441069567762, -346.4990941667554125 ) ) ;
#64940=CARTESIAN_POINT ( 'NONE',  ( 3.599051426031238066, -281.2830818832589443, -331.3404451276120426 ) ) ;
#64941=CARTESIAN_POINT ( 'NONE',  ( -112.2774090673670173, -280.5124506605142187, -273.4659805666461807 ) ) ;
#64942=CARTESIAN_POINT ( 'NONE',  ( -112.4437553364018214, -272.9313224066769408, -253.3704938614554862 ) ) ;
#64943=CARTESIAN_POINT ( 'NONE',  ( 3.499701719940560452, -276.3527600724881950, -335.7000626932079967 ) ) ;
#64944=CARTESIAN_POINT ( 'NONE',  ( -3.663725490660570738, -296.5243944182886935, -336.7614487047821399 ) ) ;
#64948=CARTESIAN_POINT ( 'NONE',  ( -58.52898931017722362, -293.4626745613730350, -343.1578428536843148 ) ) ;
#64949=CARTESIAN_POINT ( 'NONE',  ( -19.25032703536248135, -273.7987968974132968, -199.5224133838598846 ) ) ;
#64950=CARTESIAN_POINT ( 'NONE',  ( -11.40726733078074950, -293.9039586015770738, -198.5413036611478788 ) ) ;
#64951=CARTESIAN_POINT ( 'NONE',  ( -37.30987171927208124, -279.5519495502701943, -345.3611179825600175 ) ) ;
#64952=CARTESIAN_POINT ( 'NONE',  ( -1.005805344258491107, -293.7286398533959755, -202.9243960164357929 ) ) ;
#64953=CARTESIAN_POINT ( 'NONE',  ( -87.95096575868657851, -291.7615039333078926, -325.5560745152930053 ) ) ;
#64954=CARTESIAN_POINT ( 'NONE',  ( -110.0654507216758304, -276.7790754417439416, -252.7178606251402755 ) ) ;
#64955=CARTESIAN_POINT ( 'NONE',  ( -72.30940717321766442, -279.4386687504831457, -336.0913492280743640 ) ) ;
#64956=CARTESIAN_POINT ( 'NONE',  ( -20.54659779827102994, -292.9147970178929086, -342.9348551313277085 ) ) ;
#64957=CARTESIAN_POINT ( 'NONE',  ( 21.00409251012510126, -282.7521936363731925, -222.0281689178572435 ) ) ;
#64958=CARTESIAN_POINT ( 'NONE',  ( -96.17801707996994764, -282.8616657493402613, -314.0934159086996829 ) ) ;
#64960=CARTESIAN_POINT ( 'NONE',  ( -95.94124855122180406, -283.6079352944829566, -313.9292303062280780 ) ) ;
#64961=CARTESIAN_POINT ( 'NONE',  ( -17.08691519550920290, -281.3873889154195354, -196.3933128490536717 ) ) ;
#64962=CARTESIAN_POINT ( 'NONE',  ( -97.74086255970986770, -282.7143024068138857, -317.4774622581012409 ) ) ;
#64963=CARTESIAN_POINT ( 'NONE',  ( -110.4389182992568124, -279.1957884895527400, -293.9760891873529545 ) ) ;
#64964=( LENGTH_UNIT ( ) NAMED_UNIT ( * ) SI_UNIT ( .MILLI., .METRE. ) );
#64965=CARTESIAN_POINT ( 'NONE',  ( -17.51918670569879311, -278.3210280942863619, -344.0481298137309523 ) ) ;
#64966=CARTESIAN_POINT ( 'NONE',  ( -67.68488546085839630, -297.9805209788416391, -333.4427485647536855 ) ) ;
#64969=CARTESIAN_POINT ( 'NONE',  ( -91.50745806583132946, -299.2815941995204980, -218.4112298104505498 ) ) ;
#64970=CARTESIAN_POINT ( 'NONE',  ( -92.19326688385801560, -275.8605346611529399, -321.0639181143576479 ) ) ;
#64971=CARTESIAN_POINT ( 'NONE',  ( -98.40384439313966425, -292.9217435012909050, -225.1133407510679092 ) ) ;
#64972=CARTESIAN_POINT ( 'NONE',  ( 35.00981012005320281, -292.7631073201330878, -259.9135520915473307 ) ) ;
#64973=CARTESIAN_POINT ( 'NONE',  ( -31.83744570529959717, -288.4922379185161958, -347.1549512748050574 ) ) ;
#64975=CARTESIAN_POINT ( 'NONE',  ( 27.59552342027188487, -292.6587633879446457, -310.7316096564471763 ) ) ;
#64976=CARTESIAN_POINT ( 'NONE',  ( -5.434517483399896598, -284.8788800529824812, -203.8011664787330517 ) ) ;
#64977=CARTESIAN_POINT ( 'NONE',  ( -93.50628927240444455, -293.0927038958209323, -221.8183079224989456 ) ) ;
#64978=CARTESIAN_POINT ( 'NONE',  ( -67.97475640748461956, -284.7781563470576316, -337.1657536181999717 ) ) ;
#64979=CARTESIAN_POINT ( 'NONE',  ( -31.83166314781207262, -289.9256057536100002, -346.9802141575967767 ) ) ;
#64980=CARTESIAN_POINT ( 'NONE',  ( -9.229457628856597040, -280.9222438678889375, -202.9245532462947779 ) ) ;
#64981=CARTESIAN_POINT ( 'NONE',  ( 37.39312980538593223, -292.5591998034622634, -287.2343709391707307 ) ) ;
#64982=CARTESIAN_POINT ( 'NONE',  ( -45.99740481066345410, -289.9619579705826595, -346.7635770091013114 ) ) ;
#64983=CARTESIAN_POINT ( 'NONE',  ( -110.7212541379692965, -290.7516360884237656, -293.6644971242484417 ) ) ;
#64984=CARTESIAN_POINT ( 'NONE',  ( -41.32505135933491403, -286.1673207976138542, -197.4573793176499521 ) ) ;
#64985=VERTEX_POINT ( 'NONE', #26036 ) ;
#64987=CARTESIAN_POINT ( 'NONE',  ( 21.34514669769989936, -296.0664174347120934, -318.2997516510645823 ) ) ;
#64988=CARTESIAN_POINT ( 'NONE',  ( -113.8446720159697065, -295.2466769315292936, -269.5906871005794301 ) ) ;
#64989=CARTESIAN_POINT ( 'NONE',  ( -108.8338383194471248, -277.8204406134950091, -254.4203464208620744 ) ) ;
#64990=CARTESIAN_POINT ( 'NONE',  ( -110.9763953039622493, -272.3420635680531063, -247.8752727268632725 ) ) ;
#64991=CIRCLE ( 'NONE', #30139, 5.343514653206204557 ) ;
#64992=CARTESIAN_POINT ( 'NONE',  ( -26.12075352961271335, -293.3865705447582855, -343.1951629649485653 ) ) ;
#64993=CARTESIAN_POINT ( 'NONE',  ( 36.61569684423406557, -277.3641370944048958, -274.3451360666684877 ) ) ;
#64994=CARTESIAN_POINT ( 'NONE',  ( -46.30481724080509309, -272.0768071443362146, -196.6690016424053908 ) ) ;
#64995=CARTESIAN_POINT ( 'NONE',  ( 20.48630558546545544, -294.1233050671763181, -225.1406403916678869 ) ) ;
#64996=CARTESIAN_POINT ( 'NONE',  ( -98.98580949401275575, -297.0839198735492346, -310.1306523387345919 ) ) ;
#64998=CARTESIAN_POINT ( 'NONE',  ( -91.39672056065612082, -293.8190723162027211, -322.5921738032370172 ) ) ;
#65000=CARTESIAN_POINT ( 'NONE',  ( -68.14425835412929189, -298.3097102831461598, -199.8450762957822633 ) ) ;
#65001=CARTESIAN_POINT ( 'NONE',  ( -93.53304422316939792, -275.2430403383432918, -220.6868439636174912 ) ) ;
#65002=CARTESIAN_POINT ( 'NONE',  ( -110.5721908646213052, -291.4823795916028075, -271.1999706868085696 ) ) ;
#65003=CARTESIAN_POINT ( 'NONE',  ( -15.58248214811220222, -295.0960941066388727, -340.1181356406543159 ) ) ;
#65004=CARTESIAN_POINT ( 'NONE',  ( -97.28365527322517892, -281.1542781798481201, -224.6742512743268207 ) ) ;
#65005=CARTESIAN_POINT ( 'NONE',  ( -35.33208881341227681, -278.7616817725262877, -193.8676121899182760 ) ) ;
#65007=CARTESIAN_POINT ( 'NONE',  ( -67.84855252307130513, -282.7907836758585631, -340.9489692303662309 ) ) ;
#65008=CARTESIAN_POINT ( 'NONE',  ( 35.63585796778031067, -274.5933015986652208, -245.9529804386882859 ) ) ;
#65009=CARTESIAN_POINT ( 'NONE',  ( -102.7146785439990140, -277.4690871465581949, -231.1073970538200228 ) ) ;
#65010=CARTESIAN_POINT ( 'NONE',  ( 20.57479640587767378, -278.8922418235802638, -222.4475723026494620 ) ) ;
#65012=CARTESIAN_POINT ( 'NONE',  ( -55.39873258125298605, -296.4998840667466311, -199.0681103036263835 ) ) ;
#65013=CARTESIAN_POINT ( 'NONE',  ( 9.701507942140940699, -276.6992781592539359, -211.8834195356988346 ) ) ;
#65015=CARTESIAN_POINT ( 'NONE',  ( 23.50164100436456849, -290.9691743327213658, -225.9033330078058270 ) ) ;
#65016=CARTESIAN_POINT ( 'NONE',  ( -89.49148258356979113, -289.7631774190076044, -327.0126862736960902 ) ) ;
#65017=CARTESIAN_POINT ( 'NONE',  ( -8.420109569228346302, -276.4298878480741450, -200.9259816152268741 ) ) ;
#65018=CARTESIAN_POINT ( 'NONE',  ( -40.57224733803614924, -296.0112990370118951, -195.5846799292339426 ) ) ;
#65019=CARTESIAN_POINT ( 'NONE',  ( -76.01658475944793736, -284.7468072085644621, -203.9039765725950986 ) ) ;
#65020=CARTESIAN_POINT ( 'NONE',  ( -112.3924214805754360, -282.5558719554007325, -270.0585568334979030 ) ) ;
#65022=CARTESIAN_POINT ( 'NONE',  ( 23.67985290077372795, -291.7837456107552612, -229.5750839650057173 ) ) ;
#65023=CARTESIAN_POINT ( 'NONE',  ( -75.33222439773294354, -283.6794072767269199, -206.5834922356388574 ) ) ;
#65026=CARTESIAN_POINT ( 'NONE',  ( 26.56504906341792349, -291.0241908038734664, -231.0078170028048703 ) ) ;
#65027=CARTESIAN_POINT ( 'NONE',  ( -95.75219581073891106, -282.3647043226262099, -319.4824796599507977 ) ) ;
#65028=CARTESIAN_POINT ( 'NONE',  ( -93.32029419791268765, -279.4749640461055264, -318.4530863628002066 ) ) ;
#65029=CARTESIAN_POINT ( 'NONE',  ( -40.81391583870370710, -287.2145928977079166, -193.7849995979883033 ) ) ;
#65030=CARTESIAN_POINT ( 'NONE',  ( -7.016504831150768062, -286.4614861796586638, -203.9442095719910810 ) ) ;
#65031=CARTESIAN_POINT ( 'NONE',  ( -95.72954365407453281, -279.3522802100104059, -315.1521287678070280 ) ) ;
#65032=CARTESIAN_POINT ( 'NONE',  ( -110.1278571766150378, -279.4588069847839620, -262.4737467759662195 ) ) ;
#65033=CARTESIAN_POINT ( 'NONE',  ( -112.3281035586150409, -286.5925953445448613, -267.2241425472863057 ) ) ;
#65035=CARTESIAN_POINT ( 'NONE',  ( -40.43813179861543006, -297.8476904058522337, -193.3712755926543707 ) ) ;
#65036=CARTESIAN_POINT ( 'NONE',  ( 30.93962469985678965, -289.9304453970094642, -300.6474983243394377 ) ) ;
#65038=CARTESIAN_POINT ( 'NONE',  ( -55.56934967048406548, -279.7662352645559736, -350.3683826091709648 ) ) ;
#65040=CARTESIAN_POINT ( 'NONE',  ( 33.69823470673961197, -292.3049112733814923, -297.9250087201768338 ) ) ;
#65041=CARTESIAN_POINT ( 'NONE',  ( -4.300892196741418871, -288.0160145898828432, -204.4899348624456650 ) ) ;
#65042=CARTESIAN_POINT ( 'NONE',  ( 34.31008639629446577, -283.5543844227261729, -288.9587766495695291 ) ) ;
#65043=CARTESIAN_POINT ( 'NONE',  ( 33.30764423547869768, -288.6030906802274103, -241.1149580787556488 ) ) ;
#65044=CARTESIAN_POINT ( 'NONE',  ( -4.529283412413871446, -289.9439969738307923, -339.4887728749631606 ) ) ;
#65045=CARTESIAN_POINT ( 'NONE',  ( -111.3999709160549827, -286.7054854849619119, -258.4316797885995243 ) ) ;
#65046=CARTESIAN_POINT ( 'NONE',  ( -114.2318936896619306, -278.6674214187959819, -274.4718525336907646 ) ) ;
#65048=CARTESIAN_POINT ( 'NONE',  ( 37.38868045229116888, -291.7743100003077075, -281.5273356325625400 ) ) ;
#65049=CARTESIAN_POINT ( 'NONE',  ( 36.60031376267445324, -281.1155184187628038, -248.8294644994108467 ) ) ;
#65050=CARTESIAN_POINT ( 'NONE',  ( -88.19644433264322458, -275.1919163534752215, -216.2105846099405255 ) ) ;
#65052=CARTESIAN_POINT ( 'NONE',  ( -69.91165696735023971, -294.1233781216987495, -202.8022627189028810 ) ) ;
#65054=CARTESIAN_POINT ( 'NONE',  ( -31.31774836845783838, -272.3670796898460367, -194.6004963957727227 ) ) ;
#65056=CARTESIAN_POINT ( 'NONE',  ( -9.217869101949890620, -279.9377085392704885, -202.9293853177581184 ) ) ;
#65057=CARTESIAN_POINT ( 'NONE',  ( 32.18618075494870112, -276.3422755766988530, -238.0808119201695376 ) ) ;
#65059=CARTESIAN_POINT ( 'NONE',  ( -94.07940219535004189, -298.6366098499015038, -223.4777913896885764 ) ) ;
#65060=CARTESIAN_POINT ( 'NONE',  ( -10.79468827121161212, -281.7731639034983004, -342.4458900911664614 ) ) ;
#65061=CARTESIAN_POINT ( 'NONE',  ( -110.9833490451023295, -292.4086881721431723, -262.9529092179504346 ) ) ;
#65062=CARTESIAN_POINT ( 'NONE',  ( -87.02563648856381917, -298.8954524125682610, -212.3758685898957594 ) ) ;
#65064=CARTESIAN_POINT ( 'NONE',  ( -107.4160447862182224, -298.1555591537640453, -239.2848801264625536 ) ) ;
#65066=CARTESIAN_POINT ( 'NONE',  ( -36.96127528485158109, -297.0475027567128450, -345.2062253746649390 ) ) ;
#65067=CARTESIAN_POINT ( 'NONE',  ( -94.84683218277757533, -281.8891917127844522, -318.2483628126325357 ) ) ;
#65068=CARTESIAN_POINT ( 'NONE',  ( -112.9033874417387722, -290.4036621701820877, -255.5895546998198142 ) ) ;
#65069=CARTESIAN_POINT ( 'NONE',  ( -18.84009304870927082, -272.3114912752647570, -197.9919650025553324 ) ) ;
#65070=CARTESIAN_POINT ( 'NONE',  ( -5.130836386093802659, -288.0692251549377261, -201.3038904441487205 ) ) ;
#65071=CARTESIAN_POINT ( 'NONE',  ( -105.9953054164847543, -289.8157181324237399, -244.5090069921172358 ) ) ;
#65072=CARTESIAN_POINT ( 'NONE',  ( 203.6388754965839496, 292.3982009288597510, -83.13072119195177834 ) ) ;
#65073=EDGE_LOOP ( 'NONE', ( #59613, #35353, #49189, #78344 ) ) ;
#65074=CARTESIAN_POINT ( 'NONE',  ( -108.9154855428094208, -289.4695772829470002, -243.4559990169177865 ) ) ;
#65075=CARTESIAN_POINT ( 'NONE',  ( -15.84947658711131169, -288.4332023146716324, -340.2005736601225863 ) ) ;
#65077=CARTESIAN_POINT ( 'NONE',  ( -91.69365165870306100, -286.3789648975975979, -216.2560546872649354 ) ) ;
#65078=CARTESIAN_POINT ( 'NONE',  ( -72.84857431343088763, -277.8696201891085025, -334.1826298475584736 ) ) ;
#65079=CARTESIAN_POINT ( 'NONE',  ( 38.50878463611227431, -292.6146570230254724, -281.6835060179772654 ) ) ;
#65080=CARTESIAN_POINT ( 'NONE',  ( -47.23502070177807610, -283.8261319082021714, -346.6201174148558266 ) ) ;
#65081=CARTESIAN_POINT ( 'NONE',  ( -1.640176690575162910, -282.9253304198406909, -338.5604252799167284 ) ) ;
#65082=CARTESIAN_POINT ( 'NONE',  ( 34.35419165398938190, -281.7019315727233106, -256.4465613549074874 ) ) ;
#65083=CARTESIAN_POINT ( 'NONE',  ( -113.5232974181574832, -274.0039250406831002, -284.1871152304669863 ) ) ;
#65084=CARTESIAN_POINT ( 'NONE',  ( -14.01029086911824173, -91.12319595120793281, -359.2282198501130210 ) ) ;
#65085=CARTESIAN_POINT ( 'NONE',  ( 43.91850979000791000, 11.98664398100423334, -328.7862006914569406 ) ) ;
#65086=CARTESIAN_POINT ( 'NONE',  ( -19.22176515920261508, -273.4883614712646249, -199.4264900984424003 ) ) ;
#65087=CARTESIAN_POINT ( 'NONE',  ( -6.386002136165075171, -273.3889597544974208, -203.9083465094957148 ) ) ;
#65088=CARTESIAN_POINT ( 'NONE',  ( -84.15273514929729970, -295.1837198053062821, -331.4877232771656281 ) ) ;
#65089=CARTESIAN_POINT ( 'NONE',  ( 174.4399942972555664, 240.3132199972240812, -177.3433689288450239 ) ) ;
#65090=CARTESIAN_POINT ( 'NONE',  ( -96.54373969401257227, -271.8920344201064268, -221.8802134396371741 ) ) ;
#65091=CARTESIAN_POINT ( 'NONE',  ( -68.58868350556366522, -299.4975491971368342, -203.0085875688419605 ) ) ;
#65092=CARTESIAN_POINT ( 'NONE',  ( 35.76323752387585131, -288.7684825108344739, -262.8171423497376509 ) ) ;
#65094=CARTESIAN_POINT ( 'NONE',  ( -92.51952278498072246, -296.7600104201015938, -323.7299112949729079 ) ) ;
#65095=CARTESIAN_POINT ( 'NONE',  ( 13.17758103872245634, -287.2736378670214776, -217.5107354965741138 ) ) ;
#65096=CARTESIAN_POINT ( 'NONE',  ( -2.684880912629829197, -273.4198537449718742, -201.9330432040923711 ) ) ;
#65097=CARTESIAN_POINT ( 'NONE',  ( 32.08850876903645144, -294.7791104785487732, -303.4033397123219515 ) ) ;
#65098=CARTESIAN_POINT ( 'NONE',  ( 11.16437903475552496, -294.8935698847126332, -330.1515266224271841 ) ) ;
#65099=CARTESIAN_POINT ( 'NONE',  ( -110.3061898342085811, -290.6720034923824869, -273.9110735125584597 ) ) ;
#65101=CARTESIAN_POINT ( 'NONE',  ( -100.0278427780952626, -275.0397281648495209, -228.0807042868414669 ) ) ;
#65102=CARTESIAN_POINT ( 'NONE',  ( 37.83205994756009005, -274.1619325833966627, -255.6330999294527260 ) ) ;
#65104=CARTESIAN_POINT ( 'NONE',  ( -106.2930175166307833, -277.6193899738753430, -304.6166555712545119 ) ) ;
#65105=CARTESIAN_POINT ( 'NONE',  ( 19.62928128541905437, -273.2944252534488214, -223.4489906150918728 ) ) ;
#65106=CARTESIAN_POINT ( 'NONE',  ( -87.55500195373751637, -274.4112975495216915, -216.8795211431189784 ) ) ;
#65107=CARTESIAN_POINT ( 'NONE',  ( 34.85559791110665628, -276.3308703026121407, -258.0001815018592879 ) ) ;
#65108=CARTESIAN_POINT ( 'NONE',  ( 22.81667247092959983, -276.6842207497820709, -223.9185696319567569 ) ) ;
#65109=CARTESIAN_POINT ( 'NONE',  ( -12.43415599607835631, -274.7500484461702399, -341.5356077846250287 ) ) ;
#65110=CARTESIAN_POINT ( 'NONE',  ( -98.81453139608339598, -296.6557307269824264, -310.0137088135516592 ) ) ;
#65111=CARTESIAN_POINT ( 'NONE',  ( -18.08363902885875518, -293.3737114736645708, -341.3857756605856366 ) ) ;
#65113=CARTESIAN_POINT ( 'NONE',  ( -84.53413555049628769, -279.9145575383950586, -209.5285641413592543 ) ) ;
#65114=CARTESIAN_POINT ( 'NONE',  ( 7.582063831993099967, -276.5864368085204887, -327.9655645340899355 ) ) ;
#65115=CARTESIAN_POINT ( 'NONE',  ( -2.432881682194780737, -285.1889901072894986, -202.2680281996405540 ) ) ;
#65116=CARTESIAN_POINT ( 'NONE',  ( -102.2791239241788190, -299.0580786976456693, -232.4013933698420544 ) ) ;
#65118=CARTESIAN_POINT ( 'NONE',  ( 28.96059536483316776, -286.3326073100376448, -239.4320485042985069 ) ) ;
#65119=CARTESIAN_POINT ( 'NONE',  ( -64.72866823324253005, -275.6544579564328501, -339.1754837789096655 ) ) ;
#65120=CARTESIAN_POINT ( 'NONE',  ( -26.95615195961621069, -275.4922301760327628, -343.2138139198715407 ) ) ;
#65121=CARTESIAN_POINT ( 'NONE',  ( 7.324271778399890742, -284.4439115841490207, -330.6739603698275118 ) ) ;
#65122=CARTESIAN_POINT ( 'NONE',  ( -41.86581010639052636, -278.3154721361077009, -343.6312940505091547 ) ) ;
#65124=CARTESIAN_POINT ( 'NONE',  ( 12.16920554484783068, -274.7763778477155938, -328.2844348155628040 ) ) ;
#65126=CARTESIAN_POINT ( 'NONE',  ( 9.544111777519209028, -275.3681175020474257, -214.2090685116437498 ) ) ;
#65127=CARTESIAN_POINT ( 'NONE',  ( -5.738539955507913959, -282.4668990882411777, -202.1609075887422193 ) ) ;
#65129=CARTESIAN_POINT ( 'NONE',  ( 36.42457180151981078, -289.6816367715828733, -286.7864351565069114 ) ) ;
#65130=CARTESIAN_POINT ( 'NONE',  ( -3.883691926935517902, -290.4932518030722122, -203.2235449730465291 ) ) ;
#65133=CARTESIAN_POINT ( 'NONE',  ( -89.58101486556216742, -271.9812776523679645, -218.6668487309374882 ) ) ;
#65134=CARTESIAN_POINT ( 'NONE',  ( -77.91070366289109472, -289.6402465910668980, -208.1918214527433406 ) ) ;
#65135=CARTESIAN_POINT ( 'NONE',  ( -26.16130516772507875, -127.9538472306148122, -363.7897947155308884 ) ) ;
#65137=CARTESIAN_POINT ( 'NONE',  ( -26.26450177189316904, -287.3934725382138708, -345.8594850372799669 ) ) ;
#65138=CARTESIAN_POINT ( 'NONE',  ( -112.5990238542928807, -282.6541898128947423, -281.2363657905976311 ) ) ;
#65139=CARTESIAN_POINT ( 'NONE',  ( -32.08564707325928822, -284.4098255744436301, -343.7624042370968027 ) ) ;
#65140=CARTESIAN_POINT ( 'NONE',  ( -94.40454644069204448, -284.7091484574964397, -316.1678678109452107 ) ) ;
#65141=CARTESIAN_POINT ( 'NONE',  ( -112.7241150043125515, -292.5568186285869388, -268.4227295041262096 ) ) ;
#65142=CARTESIAN_POINT ( 'NONE',  ( -34.10833172957043047, -274.4250556067377147, -193.4501979491883787 ) ) ;
#65143=CARTESIAN_POINT ( 'NONE',  ( -84.28946036545470122, -287.7716662728972210, -329.6328064005700753 ) ) ;
#65144=CARTESIAN_POINT ( 'NONE',  ( -5.284774995942194131, -276.6418342691904968, -340.3707855369228810 ) ) ;
#65145=CARTESIAN_POINT ( 'NONE',  ( 33.35079023463672598, -295.2187334143389990, -246.2333469219663300 ) ) ;
#65147=CARTESIAN_POINT ( 'NONE',  ( -37.30987171927208124, -297.5519495502701943, -345.3611179825600175 ) ) ;
#65148=CARTESIAN_POINT ( 'NONE',  ( -64.25142883712764785, -282.0956160253958274, -338.7505175933482064 ) ) ;
#65149=CARTESIAN_POINT ( 'NONE',  ( -64.00680458375488513, -277.7043532314712593, -200.2066226660132600 ) ) ;
#65150=CARTESIAN_POINT ( 'NONE',  ( -30.55260384793811568, -296.5356852809806014, -194.1629249112967273 ) ) ;
#65151=CARTESIAN_POINT ( 'NONE',  ( 35.80068761150581480, -274.9169883601151696, -271.5949533400335554 ) ) ;
#65152=CARTESIAN_POINT ( 'NONE',  ( 17.23878343649675671, -294.3687364833986067, -220.7718707143359893 ) ) ;
#65153=CARTESIAN_POINT ( 'NONE',  ( 21.17460470564320119, -293.8769766968659383, -226.3241957769065209 ) ) ;
#65154=CARTESIAN_POINT ( 'NONE',  ( -22.32746989708762086, -293.6659271199785053, -195.3860566328398249 ) ) ;
#65155=CARTESIAN_POINT ( 'NONE',  ( 38.36141589626591042, -294.7236355228316143, -258.9455975846146885 ) ) ;
#65156=CARTESIAN_POINT ( 'NONE',  ( -105.9879126152182351, -296.0528879423655439, -295.3431607320734997 ) ) ;
#65157=CARTESIAN_POINT ( 'NONE',  ( -59.24966273850005649, -291.3357502855076859, -342.1443089059626459 ) ) ;
#65158=CARTESIAN_POINT ( 'NONE',  ( -93.43008208074299148, -283.9986009193834207, -323.1354793585153971 ) ) ;
#65159=CARTESIAN_POINT ( 'NONE',  ( -75.78521302646608149, -271.6847189406719281, -205.0134351872038394 ) ) ;
#65160=CARTESIAN_POINT ( 'NONE',  ( 26.35855866060897057, -286.8148656126384139, -227.0793037278084796 ) ) ;
#65161=CARTESIAN_POINT ( 'NONE',  ( -98.99342632410547083, -279.9594347785156288, -312.4433168352484245 ) ) ;
#65162=CARTESIAN_POINT ( 'NONE',  ( 4.870741441887367351, -285.6965666009664915, -210.4532670905252303 ) ) ;
#65163=CARTESIAN_POINT ( 'NONE',  ( -83.94245381970371511, -287.6916727200556352, -329.1927813444013964 ) ) ;
#65164=CARTESIAN_POINT ( 'NONE',  ( -113.1493912600846841, -276.6764366587346444, -271.5647438394866526 ) ) ;
#65165=CARTESIAN_POINT ( 'NONE',  ( 193.6056169066500274, 279.7126221763799094, -126.0203154767880989 ) ) ;
#65166=CARTESIAN_POINT ( 'NONE',  ( -104.1721159660569498, -283.6628130992014007, -299.8854123922799886 ) ) ;
#65167=CARTESIAN_POINT ( 'NONE',  ( 22.22424236409775844, -283.4066006951380245, -318.5472345616836947 ) ) ;
#65168=CARTESIAN_POINT ( 'NONE',  ( -8.333189791669957103, -287.7402746410861027, -341.4480244741359343 ) ) ;
#65169=CARTESIAN_POINT ( 'NONE',  ( -112.5066536882135324, -279.9940931680806671, -282.8779135936555917 ) ) ;
#65171=CARTESIAN_POINT ( 'NONE',  ( -51.20670599493102770, -278.5410160725589890, -345.6011331594845615 ) ) ;
#65172=CARTESIAN_POINT ( 'NONE',  ( -83.43609499822072451, -279.2333319198467620, -213.6890966540365753 ) ) ;
#65173=CARTESIAN_POINT ( 'NONE',  ( 1.446102869352315023, -276.5531448027190891, -206.5853142570784939 ) ) ;
#65174=CARTESIAN_POINT ( 'NONE',  ( 36.70416314821815718, -293.2868168420667416, -249.1893879345943503 ) ) ;
#65175=CARTESIAN_POINT ( 'NONE',  ( 15.22418897315582775, -286.3254863203099490, -323.3580434076228585 ) ) ;
#65177=CARTESIAN_POINT ( 'NONE',  ( -14.12974226088500806, -293.9482980068891607, -197.7271830719465413 ) ) ;
#65178=CARTESIAN_POINT ( 'NONE',  ( -92.43201502191433860, -294.7849934341749076, -318.7272557142741789 ) ) ;
#65179=CARTESIAN_POINT ( 'NONE',  ( 6.458736340335631709, -284.3719295228690953, -330.5511168226627774 ) ) ;
#65180=CARTESIAN_POINT ( 'NONE',  ( -42.39542323054588024, -294.7843599771210847, -343.2071705152927734 ) ) ;
#65182=CARTESIAN_POINT ( 'NONE',  ( -90.58128421845070477, -292.3990351916302188, -215.0874091386716884 ) ) ;
#65183=CARTESIAN_POINT ( 'NONE',  ( 33.55240461913435723, -281.9679774520059823, -252.4800128018499095 ) ) ;
#65184=CARTESIAN_POINT ( 'NONE',  ( -14.90865016549609123, -297.2471622246442848, -193.6742277851535334 ) ) ;
#65185=CARTESIAN_POINT ( 'NONE',  ( -98.94249613682718802, -290.5901195295340358, -316.4117367138375130 ) ) ;
#65186=CARTESIAN_POINT ( 'NONE',  ( -94.42004502758976514, -282.0069648683203241, -320.1844862526012889 ) ) ;
#65187=CARTESIAN_POINT ( 'NONE',  ( -103.1999545804094822, -291.4069023456658556, -230.4031657631257985 ) ) ;
#65188=CARTESIAN_POINT ( 'NONE',  ( -12.01862849265304689, -286.7243167846764322, -201.8714871636321107 ) ) ;
#65190=CARTESIAN_POINT ( 'NONE',  ( -104.7172394706867067, -254.0594188280566073, -325.1787590629403439 ) ) ;
#65191=CARTESIAN_POINT ( 'NONE',  ( -30.80187348468898278, -124.8376641225716810, -360.4214517073238540 ) ) ;
#65193=CARTESIAN_POINT ( 'NONE',  ( -107.3787478736263381, -278.0287493317208600, -249.2089627681827722 ) ) ;
#65194=CARTESIAN_POINT ( 'NONE',  ( -49.17833494354143653, -278.8180749322415295, -198.0138986226862130 ) ) ;
#65195=CARTESIAN_POINT ( 'NONE',  ( 29.93112004619106159, -274.7324711801586545, -232.8334263006657352 ) ) ;
#65196=CARTESIAN_POINT ( 'NONE',  ( -87.43311609469282075, -230.8234426471767335, -345.6592249140303466 ) ) ;
#65197=CARTESIAN_POINT ( 'NONE',  ( -84.19123524391571323, -277.9972466238668858, -209.9308771834095069 ) ) ;
#65198=CARTESIAN_POINT ( 'NONE',  ( -74.64004911659841923, -281.5707601945397300, -335.0782071112436711 ) ) ;
#65199=CARTESIAN_POINT ( 'NONE',  ( -108.9041640195071921, -298.6390941300284112, -244.8114061582887473 ) ) ;
#65200=CARTESIAN_POINT ( 'NONE',  ( -91.72315337734127638, -291.7423674553141382, -221.5505395597147924 ) ) ;
#65201=CARTESIAN_POINT ( 'NONE',  ( 23.14632853441941762, -286.8147105643434998, -312.1258601944918496 ) ) ;
#65202=CARTESIAN_POINT ( 'NONE',  ( -60.84786326694463554, -274.4064754819924019, -197.0882588120444723 ) ) ;
#65203=CARTESIAN_POINT ( 'NONE',  ( -68.04945934711490452, -297.8040878391975070, -204.1203174720320419 ) ) ;
#65206=CARTESIAN_POINT ( 'NONE',  ( -112.9376460530305479, -280.4923435262941211, -268.7890723547576499 ) ) ;
#65207=CARTESIAN_POINT ( 'NONE',  ( 17.28400562998450241, -281.9352794054693163, -221.4708495797858632 ) ) ;
#65208=CARTESIAN_POINT ( 'NONE',  ( 14.45399818341865839, -282.5284725036201507, -214.6908314395851107 ) ) ;
#65209=CARTESIAN_POINT ( 'NONE',  ( -4.733128820885818655, -281.6704210381087705, -335.9361858527531126 ) ) ;
#65210=CARTESIAN_POINT ( 'NONE',  ( -94.30205790202462879, -271.6883720718137738, -223.5843032265325405 ) ) ;
#65213=CARTESIAN_POINT ( 'NONE',  ( 36.34153287223616502, -276.6294867409338849, -292.2006793715371487 ) ) ;
#65215=CARTESIAN_POINT ( 'NONE',  ( 21.09904473890400567, -278.1992681471870128, -317.3886747927066381 ) ) ;
#65218=CARTESIAN_POINT ( 'NONE',  ( -112.1889198146302817, -286.6436728857402727, -261.6261018402218497 ) ) ;
#65219=CARTESIAN_POINT ( 'NONE',  ( 11.04524603365648971, -291.9392154306532916, -215.4181474100658988 ) ) ;
#65220=CARTESIAN_POINT ( 'NONE',  ( 31.33448909104350477, -286.4549800450564021, -235.7649647193582894 ) ) ;
#65221=CARTESIAN_POINT ( 'NONE',  ( -99.89936526694434349, -282.2517912348295113, -310.0110284162740868 ) ) ;
#65222=CARTESIAN_POINT ( 'NONE',  ( -37.56035519588864702, -281.6297034834774990, -343.9625541587451494 ) ) ;
#65223=CARTESIAN_POINT ( 'NONE',  ( -6.396000258704246377, -284.5416427496026586, -202.6442533920717040 ) ) ;
#65224=CARTESIAN_POINT ( 'NONE',  ( 18.80798210020796546, -283.4252345427393607, -317.6494779816167693 ) ) ;
#65225=CARTESIAN_POINT ( 'NONE',  ( 6.097897530510628883, -272.6409561375065778, -209.1581660333129946 ) ) ;
#65226=CARTESIAN_POINT ( 'NONE',  ( -96.56366273370623787, -282.3019913221716592, -318.3315984847617983 ) ) ;
#65227=CARTESIAN_POINT ( 'NONE',  ( -96.67617012817308364, -297.9236062913669230, -316.2350901513532335 ) ) ;
#65228=CARTESIAN_POINT ( 'NONE',  ( -38.72497260189452817, -281.0693086095133708, -345.5150599128980957 ) ) ;
#65229=CARTESIAN_POINT ( 'NONE',  ( -101.0222944009613713, -279.9871631521448876, -234.1922036964794529 ) ) ;
#65230=CARTESIAN_POINT ( 'NONE',  ( -4.318342954073128404, -288.4865236154905688, -202.8229703995945385 ) ) ;
#65233=CARTESIAN_POINT ( 'NONE',  ( 29.61140071008724917, -295.0105238006773334, -235.2257490199197889 ) ) ;
#65234=CARTESIAN_POINT ( 'NONE',  ( -43.39317789852498919, -275.1284415250990492, -345.1165877877641037 ) ) ;
#65235=CARTESIAN_POINT ( 'NONE',  ( -95.34314436489886191, -289.0666914581544233, -320.7594442174558367 ) ) ;
#65236=CARTESIAN_POINT ( 'NONE',  ( -6.448379707811984218, -293.0393336729117664, -337.3838243644204908 ) ) ;
#65237=CARTESIAN_POINT ( 'NONE',  ( -102.3005725409951623, -276.7719005310091802, -304.7353579236955738 ) ) ;
#65238=CARTESIAN_POINT ( 'NONE',  ( -63.49278125137783491, -295.8474215252201134, -200.8302244428391532 ) ) ;
#65239=CARTESIAN_POINT ( 'NONE',  ( -88.28441468808671289, -292.6359381462440865, -217.3182943505541118 ) ) ;
#65240=CARTESIAN_POINT ( 'NONE',  ( 31.98288692825981272, -278.4805209788416960, -303.7098442033570223 ) ) ;
#65241=CARTESIAN_POINT ( 'NONE',  ( -37.70528027253799053, -293.5364763835182202, -346.6798812815856650 ) ) ;
#65242=CARTESIAN_POINT ( 'NONE',  ( -95.56931727681921984, -291.5201046115790291, -315.7244980839562345 ) ) ;
#65243=CARTESIAN_POINT ( 'NONE',  ( -102.3373091727066679, -289.3138171906371667, -230.8954603941162986 ) ) ;
#65244=CARTESIAN_POINT ( 'NONE',  ( 32.88132104499118213, -289.2686986845671981, -292.5331746625878964 ) ) ;
#65246=CARTESIAN_POINT ( 'NONE',  ( -74.78979084820221601, -290.3672994908432088, -333.2267886346736532 ) ) ;
#65248=CARTESIAN_POINT ( 'NONE',  ( 9.994689702989733249, -289.6217089147236265, -330.6554725855314132 ) ) ;
#65249=CARTESIAN_POINT ( 'NONE',  ( -36.73981503967894469, -278.0797941285628667, -194.9955501459691902 ) ) ;
#65250=CARTESIAN_POINT ( 'NONE',  ( -99.41333535821576106, -279.4904923352523838, -224.8102370885552546 ) ) ;
#65252=CARTESIAN_POINT ( 'NONE',  ( -8.050863683924232461, -282.3456749241018429, -341.6060604817206467 ) ) ;
#65253=CARTESIAN_POINT ( 'NONE',  ( 18.39350502213383720, -284.8524379805000990, -220.1564059311868391 ) ) ;
#65255=CARTESIAN_POINT ( 'NONE',  ( 30.10467596667838208, -279.2788590299093130, -239.2241039801153022 ) ) ;
#65256=CARTESIAN_POINT ( 'NONE',  ( -77.43133059580873123, -283.5141286244143544, -206.9748246967708951 ) ) ;
#65258=CARTESIAN_POINT ( 'NONE',  ( -110.0123771794569620, -276.7348115156170252, -293.8054116256126349 ) ) ;
#65259=CARTESIAN_POINT ( 'NONE',  ( -78.34553825622769807, -284.4344693475500776, -205.5523395024503372 ) ) ;
#65260=CARTESIAN_POINT ( 'NONE',  ( -48.91102973045033053, -274.7039797872561167, -198.0688979670926528 ) ) ;
#65261=CARTESIAN_POINT ( 'NONE',  ( -94.92781295653404072, -292.7976773254404748, -224.1860736833043859 ) ) ;
#65262=CARTESIAN_POINT ( 'NONE',  ( -96.49158625621031149, -274.6320366496418046, -221.9682102769503445 ) ) ;
#65263=CARTESIAN_POINT ( 'NONE',  ( 32.08324031743266858, -274.9166887491608691, -247.5651547900818059 ) ) ;
#65264=CARTESIAN_POINT ( 'NONE',  ( -89.88532584151985816, -297.7936146557994448, -323.9520009522315149 ) ) ;
#65265=CARTESIAN_POINT ( 'NONE',  ( -48.86690013912242847, -289.3616203337568322, -346.5476423584430563 ) ) ;
#65266=CARTESIAN_POINT ( 'NONE',  ( 34.23693760936082953, -279.9445444868468371, -294.7271313253883136 ) ) ;
#65267=CARTESIAN_POINT ( 'NONE',  ( 34.46359639662605190, -293.0316000634022089, -242.4108932434071164 ) ) ;
#65269=CARTESIAN_POINT ( 'NONE',  ( -28.06469952927296418, -291.2313997091950455, -197.6648636932714282 ) ) ;
#65270=CARTESIAN_POINT ( 'NONE',  ( -68.71512544582297721, -293.4643346632063867, -338.4979271635406803 ) ) ;
#65273=CARTESIAN_POINT ( 'NONE',  ( -87.96871709012607710, -290.8287080751878193, -217.6139481118029266 ) ) ;
#65275=CARTESIAN_POINT ( 'NONE',  ( -85.37503908990142065, -286.3477934072787434, -210.4810832426212244 ) ) ;
#65276=CARTESIAN_POINT ( 'NONE',  ( -67.68488546085839630, -277.1237833571632905, -207.2794874003663779 ) ) ;
#65277=CARTESIAN_POINT ( 'NONE',  ( -8.487635440209615467, -293.7424562988702519, -341.5529492560272615 ) ) ;
#65278=CARTESIAN_POINT ( 'NONE',  ( -110.6307208814372416, -285.5895087055593535, -292.3614778708202380 ) ) ;
#65279=CARTESIAN_POINT ( 'NONE',  ( -108.0937498912920205, -284.1482066015774990, -288.3374206845554681 ) ) ;
#65280=CARTESIAN_POINT ( 'NONE',  ( -10.98818745746989123, -278.2223672120250626, -339.1811740889316980 ) ) ;
#65281=CARTESIAN_POINT ( 'NONE',  ( -17.81395034317745996, -292.8191808624181931, -342.4063384220154944 ) ) ;
#65282=CARTESIAN_POINT ( 'NONE',  ( 28.06391368486297111, -295.7790183553920542, -305.1128627020493127 ) ) ;
#65283=CARTESIAN_POINT ( 'NONE',  ( 33.62220002145524234, -274.5932161043384667, -289.1029263621664995 ) ) ;
#65286=CARTESIAN_POINT ( 'NONE',  ( 17.54349167034347801, -293.9607932386921334, -324.4124800443496497 ) ) ;
#65287=CARTESIAN_POINT ( 'NONE',  ( 35.10812308401312265, -289.6935031966906990, -287.4589926538305349 ) ) ;
#65288=CARTESIAN_POINT ( 'NONE',  ( -62.87401853368009341, -295.7197317415770499, -199.7869639662973782 ) ) ;
#65289=CARTESIAN_POINT ( 'NONE',  ( -90.48791314293045218, -296.8629919621058093, -325.7241135776966416 ) ) ;
#65291=CARTESIAN_POINT ( 'NONE',  ( -6.981729361334126693, -287.1127940008456108, -203.8480131727205276 ) ) ;
#65292=CARTESIAN_POINT ( 'NONE',  ( -113.9752608163959877, -277.6671682581188634, -265.8758544900713332 ) ) ;
#65293=CARTESIAN_POINT ( 'NONE',  ( -39.09718666489686711, -295.7250506077480736, -347.2391451034936836 ) ) ;
#65294=CARTESIAN_POINT ( 'NONE',  ( -4.884056993510368372, -286.7689211001621175, -338.8356203455598461 ) ) ;
#65295=CARTESIAN_POINT ( 'NONE',  ( -34.85107514289681774, -295.3549434226244443, -347.2996718991996659 ) ) ;
#65296=CARTESIAN_POINT ( 'NONE',  ( -103.5772793547167510, -291.3002529119239057, -239.6213142878302165 ) ) ;
#65299=CARTESIAN_POINT ( 'NONE',  ( 139.3042675124528103, 178.0593506815302192, -238.4361927325643080 ) ) ;
#65300=CARTESIAN_POINT ( 'NONE',  ( 34.19743212384639719, -288.7335508957171442, -243.8119125668313529 ) ) ;
#65301=CARTESIAN_POINT ( 'NONE',  ( 44.71564893372296723, -291.0523547857347353, -270.3937649182068412 ) ) ;
#65303=CARTESIAN_POINT ( 'NONE',  ( -88.85700406090930414, -278.6992749847294135, -213.2692074608133339 ) ) ;
#65304=CARTESIAN_POINT ( 'NONE',  ( -3.987709938743091875, -284.6113574507634212, -337.3502198503776413 ) ) ;
#65305=CARTESIAN_POINT ( 'NONE',  ( -109.4154064952325740, -283.4494917522649189, -244.9842162286564644 ) ) ;
#65306=CARTESIAN_POINT ( 'NONE',  ( 26.92719267051030840, -286.1388005868269602, -308.0238995172038017 ) ) ;
#65307=CARTESIAN_POINT ( 'NONE',  ( 37.51911326793244683, -277.5650742851277641, -282.3599795284450806 ) ) ;
#65308=CARTESIAN_POINT ( 'NONE',  ( -110.3027966657351868, -296.9940245040288005, -274.1908481967466855 ) ) ;
#65311=CARTESIAN_POINT ( 'NONE',  ( -35.65598151951728312, -293.7154211559209216, -343.8475160310974275 ) ) ;
#65312=CARTESIAN_POINT ( 'NONE',  ( -33.92810822136723203, -280.7454502061456196, -193.5388544315613899 ) ) ;
#65313=CARTESIAN_POINT ( 'NONE',  ( -72.84200492444578856, -277.5363928325469374, -334.1620842169902517 ) ) ;
#65314=CARTESIAN_POINT ( 'NONE',  ( -70.98120153764955376, -278.9445994371603206, -205.4449574988954907 ) ) ;
#65315=CARTESIAN_POINT ( 'NONE',  ( 25.06731933576267579, -276.0387618071033557, -225.7672903536730189 ) ) ;
#65316=CARTESIAN_POINT ( 'NONE',  ( -72.71040477222277332, -276.4297021520570752, -338.4238882509869768 ) ) ;
#65317=CARTESIAN_POINT ( 'NONE',  ( 165.9745577554829197, 231.6962457589320081, -190.8271905442535967 ) ) ;
#65318=CARTESIAN_POINT ( 'NONE',  ( -83.81235696716545647, -297.1010307119714753, -331.0832728325123639 ) ) ;
#65319=CARTESIAN_POINT ( 'NONE',  ( -54.42813229853333468, -279.7662352645560304, -345.3683826091709648 ) ) ;
#65321=CARTESIAN_POINT ( 'NONE',  ( 133.0872704186301405, -299.5541904835127980, -189.7068768330456123 ) ) ;
#65322=MECHANICAL_DESIGN_GEOMETRIC_PRESENTATION_REPRESENTATION('',(#53240),#13939);
#65323=CARTESIAN_POINT ( 'NONE',  ( -103.7713686059891103, -286.0501616071703097, -239.2354874074904103 ) ) ;
#65324=CARTESIAN_POINT ( 'NONE',  ( -66.81695248463182679, -287.4313318652025373, -200.3241026729481575 ) ) ;
#65325=CARTESIAN_POINT ( 'NONE',  ( 25.77988533533015669, -287.4073371202152885, -307.3333584263721150 ) ) ;
#65326=CARTESIAN_POINT ( 'NONE',  ( 13.63532040421435809, -281.8683679172942220, -328.0590206876794923 ) ) ;
#65328=CARTESIAN_POINT ( 'NONE',  ( -108.3829322212403241, -277.2139407260935400, -250.3247359912301704 ) ) ;
#65329=CARTESIAN_POINT ( 'NONE',  ( -107.3304754579055640, -286.0869041655930687, -295.2615113610546587 ) ) ;
#65330=CARTESIAN_POINT ( 'NONE',  ( -79.43519188038939660, -277.9519408077896969, -209.8727248557343898 ) ) ;
#65331=CARTESIAN_POINT ( 'NONE',  ( -29.64523733348267953, -278.2679838115481630, -343.5014096827242156 ) ) ;
#65332=CARTESIAN_POINT ( 'NONE',  ( 32.95878180429987481, -276.3078446760085285, -290.3024096635724618 ) ) ;
#65333=CARTESIAN_POINT ( 'NONE',  ( -15.08237165917536515, -287.5651763040362425, -343.7141293351393756 ) ) ;
#65335=CARTESIAN_POINT ( 'NONE',  ( -93.30690372224447060, -284.6346508238265756, -323.0307112219816759 ) ) ;
#65336=CARTESIAN_POINT ( 'NONE',  ( 6.894755563222777717, -282.9605139220510637, -333.3759554415153730 ) ) ;
#65340=CARTESIAN_POINT ( 'NONE',  ( 9.483457504974088792, -290.2769436734733404, -329.9905349023028975 ) ) ;
#65341=CARTESIAN_POINT ( 'NONE',  ( -112.0871577655630631, -289.0315367282999546, -286.6833371162832123 ) ) ;
#65342=CARTESIAN_POINT ( 'NONE',  ( -109.3588762503709688, -271.7893684176930833, -256.7884039423370268 ) ) ;
#65343=CARTESIAN_POINT ( 'NONE',  ( 24.73707529807938954, -292.2974386107674718, -224.9789802143407940 ) ) ;
#65344=CARTESIAN_POINT ( 'NONE',  ( -109.6225427432049884, -288.8435428208294411, -284.7849789324421295 ) ) ;
#65345=CARTESIAN_POINT ( 'NONE',  ( 33.40795021036746704, -288.5004923088713440, -250.8260857948762066 ) ) ;
#65346=CARTESIAN_POINT ( 'NONE',  ( 39.58706461736021254, -290.0519495502703080, -270.3284710469133074 ) ) ;
#65347=CARTESIAN_POINT ( 'NONE',  ( 36.15364725900674614, -289.7442375073393350, -285.3088457246223584 ) ) ;
#65348=CARTESIAN_POINT ( 'NONE',  ( -97.71646255462998454, -289.1620496503210802, -225.5632716339396495 ) ) ;
#65349=CARTESIAN_POINT ( 'NONE',  ( -105.5938252097688661, -292.9617544598418704, -239.1466366034793793 ) ) ;
#65350=CARTESIAN_POINT ( 'NONE',  ( -100.5983573168092704, -284.9885127014148338, -307.2664532196525897 ) ) ;
#65351=CARTESIAN_POINT ( 'NONE',  ( 37.40023289792614491, -295.4439952151730608, -261.9062163768480787 ) ) ;
#65354=CARTESIAN_POINT ( 'NONE',  ( -75.61943636027299931, -275.5244075809591777, -205.3914795370817785 ) ) ;
#65355=CARTESIAN_POINT ( 'NONE',  ( -18.70434817123013360, -282.0032343908314942, -341.1614331494340036 ) ) ;
#65356=CARTESIAN_POINT ( 'NONE',  ( -109.3182940398453411, -282.2800102402512721, -291.4871252058547952 ) ) ;
#65357=CARTESIAN_POINT ( 'NONE',  ( -114.1763943722265680, -295.7589359101915534, -269.5939280421946478 ) ) ;
#65358=CARTESIAN_POINT ( 'NONE',  ( 27.53542775735564518, -273.3108473875230402, -234.6321674303209477 ) ) ;
#65359=CARTESIAN_POINT ( 'NONE',  ( -104.6618806824832575, -277.0543968831531174, -238.4704458353679399 ) ) ;
#65360=CARTESIAN_POINT ( 'NONE',  ( -37.84257380046856412, -299.3609248413384307, -196.8696721863768744 ) ) ;
#65361=CARTESIAN_POINT ( 'NONE',  ( -41.14513951141092463, -272.5800319411375199, -193.9932032119276926 ) ) ;
#65362=CARTESIAN_POINT ( 'NONE',  ( -36.97452510621791077, -296.4727076717618388, -343.9619577581739236 ) ) ;
#65363=CARTESIAN_POINT ( 'NONE',  ( 82.64890176555634582, -299.5541904835127980, -197.2570935515975918 ) ) ;
#65364=CARTESIAN_POINT ( 'NONE',  ( 8.336942482371544116, -295.2116025256293028, -327.5757169327271185 ) ) ;
#65366=CARTESIAN_POINT ( 'NONE',  ( -112.5681479059690986, -282.5055862939886993, -275.5782373613286609 ) ) ;
#65367=CARTESIAN_POINT ( 'NONE',  ( -90.40723577949991352, -295.8293950681012348, -320.5642352078342583 ) ) ;
#65368=CARTESIAN_POINT ( 'NONE',  ( -112.5250916142391588, -284.3442083940905718, -286.9881334886314335 ) ) ;
#65369=CARTESIAN_POINT ( 'NONE',  ( 36.76290506810964587, -287.4806353782450401, -291.2481577722910515 ) ) ;
#65370=CARTESIAN_POINT ( 'NONE',  ( 3.255966963356850208, -290.5984256847651181, -207.4359178264753893 ) ) ;
#65371=CARTESIAN_POINT ( 'NONE',  ( -88.81568146028622834, -278.5478799972228217, -213.3121209197132941 ) ) ;
#65372=CARTESIAN_POINT ( 'NONE',  ( -110.4683760289727132, -281.8380690714489560, -287.0191576251351080 ) ) ;
#65374=CARTESIAN_POINT ( 'NONE',  ( 28.01868723161029706, -285.8945006358876526, -236.8551474084490280 ) ) ;
#65375=CARTESIAN_POINT ( 'NONE',  ( -57.22407212948342448, -288.2230547760084391, -344.4847823251547538 ) ) ;
#65378=CARTESIAN_POINT ( 'NONE',  ( -107.4733429672123890, -298.4558471392887782, -247.2208665155737890 ) ) ;
#65379=CARTESIAN_POINT ( 'NONE',  ( -84.21986526421866870, -280.8473325187399041, -209.9530847315107849 ) ) ;
#65380=CARTESIAN_POINT ( 'NONE',  ( -112.6644134575226133, -294.6179247553872642, -266.7875873619102549 ) ) ;
#65381=CARTESIAN_POINT ( 'NONE',  ( 33.34290817062729673, -281.4613005348429056, -288.7350392704406659 ) ) ;
#65382=CARTESIAN_POINT ( 'NONE',  ( 26.51292985971861782, -294.2857643577708586, -313.3911799582067488 ) ) ;
#65383=CARTESIAN_POINT ( 'NONE',  ( -64.05444240837543646, -281.7040289382188121, -200.2247446144436367 ) ) ;
#65385=CARTESIAN_POINT ( 'NONE',  ( -107.8325320897626227, -295.3492011492169809, -290.2219099575742121 ) ) ;
#65386=AXIS2_PLACEMENT_3D ( 'NONE', #46076, #2074, #67874 ) ;
#65389=CARTESIAN_POINT ( 'NONE',  ( -4.071915125946985903, -284.5910924343277770, -337.1815356145591522 ) ) ;
#65390=CARTESIAN_POINT ( 'NONE',  ( 82.17440492340898572, -297.5479941798179766, -195.4018648718562758 ) ) ;
#65391=CARTESIAN_POINT ( 'NONE',  ( -95.95921662488163406, -282.6952119285918457, -223.5744983911110353 ) ) ;
#65392=CARTESIAN_POINT ( 'NONE',  ( -5.172536408195755442, -273.6620643650621219, -200.5807215467368394 ) ) ;
#65393=CARTESIAN_POINT ( 'NONE',  ( -101.1226439263710546, -290.8722681356970270, -234.7468604560795313 ) ) ;
#65395=CARTESIAN_POINT ( 'NONE',  ( 30.65384604593693751, -282.6947087488522357, -241.9478560911747991 ) ) ;
#65396=CARTESIAN_POINT ( 'NONE',  ( -19.09330153368558669, -275.8909357807982019, -198.7998241819788632 ) ) ;
#65397=CARTESIAN_POINT ( 'NONE',  ( -5.768207181670216954, -284.2440025502988306, -339.7120729934683254 ) ) ;
#65398=CARTESIAN_POINT ( 'NONE',  ( 35.74926881489287922, -280.2521616892001362, -263.1273887159953802 ) ) ;
#65399=CARTESIAN_POINT ( 'NONE',  ( -111.8890924574281769, -280.4408017308335843, -279.0460350030853078 ) ) ;
#65400=CARTESIAN_POINT ( 'NONE',  ( 7.989098699796488567, -298.6050200815838025, -193.3611049961748733 ) ) ;
#65401=CARTESIAN_POINT ( 'NONE',  ( -32.68048220623310129, -273.9426626004316176, -193.4891809416664330 ) ) ;
#65402=CARTESIAN_POINT ( 'NONE',  ( 32.90695643179160612, -295.7954077118255896, -295.1416201410072517 ) ) ;
#65406=CARTESIAN_POINT ( 'NONE',  ( -14.18249961170248952, -292.8945004373529173, -342.4995745099487294 ) ) ;
#65407=CARTESIAN_POINT ( 'NONE',  ( -81.10285726640799453, -272.9473074455739834, -211.7916604016508018 ) ) ;
#65409=CARTESIAN_POINT ( 'NONE',  ( 31.55158653322001072, -294.6464949850137600, -237.4295049089770941 ) ) ;
#65410=CARTESIAN_POINT ( 'NONE',  ( -111.2869819898779866, -299.4805209788416391, -234.7871824221999191 ) ) ;
#65411=CARTESIAN_POINT ( 'NONE',  ( -64.26370223029951489, -292.9137546359443149, -198.5890211695690368 ) ) ;
#65412=CARTESIAN_POINT ( 'NONE',  ( -23.41972997224582187, -290.8740657442138513, -343.9410331998058155 ) ) ;
#65413=CARTESIAN_POINT ( 'NONE',  ( -111.4333763521071745, -276.6918485243790542, -259.4928026283280360 ) ) ;
#65414=CARTESIAN_POINT ( 'NONE',  ( -67.36138853243748770, -279.3691165322459824, -338.4796360849477423 ) ) ;
#65415=CARTESIAN_POINT ( 'NONE',  ( 22.46917672270312494, -292.2413821474057158, -314.6778553463686308 ) ) ;
#65416=CARTESIAN_POINT ( 'NONE',  ( 34.15408124983567717, -283.0893611010644690, -245.1314981090466176 ) ) ;
#65417=CARTESIAN_POINT ( 'NONE',  ( -100.4215314072840357, -283.7141848003756195, -307.1445704102478658 ) ) ;
#65418=CARTESIAN_POINT ( 'NONE',  ( -45.25520502765089503, -281.0339476568632904, -194.0268289148439180 ) ) ;
#65419=CARTESIAN_POINT ( 'NONE',  ( -67.02097820176535947, -284.4665939125920886, -199.7413674011825151 ) ) ;
#65420=CARTESIAN_POINT ( 'NONE',  ( -82.39846438558102193, -278.5920580619810494, -332.5118074958356829 ) ) ;
#65422=CARTESIAN_POINT ( 'NONE',  ( 30.62389622713492088, -276.6214235350834656, -235.6712712979976061 ) ) ;
#65423=CARTESIAN_POINT ( 'NONE',  ( 27.33386217378599881, -289.6233781216987495, -239.1787733560258573 ) ) ;
#65425=CARTESIAN_POINT ( 'NONE',  ( -102.3220523543144083, -275.0496087516776811, -233.1410596474597980 ) ) ;
#65426=CARTESIAN_POINT ( 'NONE',  ( -62.36443268595444778, -275.3992213541168894, -340.7418164892691834 ) ) ;
#65427=CARTESIAN_POINT ( 'NONE',  ( -111.6537581266353385, -292.5140871069919513, -254.4348366466839764 ) ) ;
#65428=CARTESIAN_POINT ( 'NONE',  ( 35.30725766619008965, -293.0136250102835334, -278.9307132030334628 ) ) ;
#65429=CARTESIAN_POINT ( 'NONE',  ( 35.79249968725556386, -286.7570320682622196, -246.2968497567650843 ) ) ;
#65431=CARTESIAN_POINT ( 'NONE',  ( -55.94453029314470882, -293.8618986950617114, -344.4727972318981415 ) ) ;
#65432=CARTESIAN_POINT ( 'NONE',  ( -65.64110728933360406, -281.8283714908260436, -338.5333883263651273 ) ) ;
#65433=CARTESIAN_POINT ( 'NONE',  ( -95.04978968866063838, -291.7630146487596221, -317.0584614092593938 ) ) ;
#65434=CARTESIAN_POINT ( 'NONE',  ( -93.77367295465313646, -283.6987636910453716, -222.9676564391809279 ) ) ;
#65435=CARTESIAN_POINT ( 'NONE',  ( -29.37465881075294760, -284.2644416329409296, -343.4720051016085449 ) ) ;
#65436=CARTESIAN_POINT ( 'NONE',  ( -85.00915919480364380, -290.6326118990021996, -330.6006312189260825 ) ) ;
#65437=CARTESIAN_POINT ( 'NONE',  ( 32.03306184477783347, -281.7386492707062757, -247.2859726534441904 ) ) ;
#65438=CARTESIAN_POINT ( 'NONE',  ( 26.17388718873376519, -292.9142299230162507, -313.1837625335593884 ) ) ;
#65439=CARTESIAN_POINT ( 'NONE',  ( 27.31446838273954114, -288.9018811909086253, -311.9771757873883189 ) ) ;
#65440=CARTESIAN_POINT ( 'NONE',  ( 37.76624037033315773, -288.2540610654318129, -287.1043363598174665 ) ) ;
#65441=CARTESIAN_POINT ( 'NONE',  ( -44.02648922586983105, -286.1319602043271857, -197.6678335663120265 ) ) ;
#65444=CARTESIAN_POINT ( 'NONE',  ( -37.65962831952445100, -296.9164669897316458, -346.1381236568839768 ) ) ;
#65445=CARTESIAN_POINT ( 'NONE',  ( -55.96654247815905592, -293.9719792569031824, -344.5663301908441554 ) ) ;
#65446=CARTESIAN_POINT ( 'NONE',  ( -81.41996954108472551, -278.4948988909398508, -211.8122817654414405 ) ) ;
#65447=CARTESIAN_POINT ( 'NONE',  ( -87.99114111674450101, -272.8738213400088739, -212.3751713304318400 ) ) ;
#65448=CARTESIAN_POINT ( 'NONE',  ( -2.836089684496048147, -293.0671690360529169, -335.4769424931977824 ) ) ;
#65449=CARTESIAN_POINT ( 'NONE',  ( 35.84028343590882315, -277.1672602316328948, -259.2138574475316091 ) ) ;
#65450=CARTESIAN_POINT ( 'NONE',  ( -34.40743603492575886, -296.3292324131429609, -196.3486720200830860 ) ) ;
#65451=CARTESIAN_POINT ( 'NONE',  ( 25.17809604026358272, -294.2289105848749386, -231.8146238006975750 ) ) ;
#65452=CARTESIAN_POINT ( 'NONE',  ( 18.21564661652627137, -295.3102711596413883, -318.2092005615400012 ) ) ;
#65454=CARTESIAN_POINT ( 'NONE',  ( -112.5329910453490925, -294.5259416621192372, -272.3941710822987829 ) ) ;
#65455=CARTESIAN_POINT ( 'NONE',  ( -106.7018606971562633, -273.7797540816976039, -237.2956231907605229 ) ) ;
#65457=CARTESIAN_POINT ( 'NONE',  ( -108.5765029324005297, -291.2698433297636598, -287.3614508714329077 ) ) ;
#65459=CARTESIAN_POINT ( 'NONE',  ( -63.57262629906725238, -295.7368371833783272, -338.5617810344954250 ) ) ;
#65460=CARTESIAN_POINT ( 'NONE',  ( -94.87668091974316553, -279.8618483902931757, -319.0444902304431594 ) ) ;
#65461=CARTESIAN_POINT ( 'NONE',  ( -113.5891559565257580, -277.1500210284460195, -277.2697733443259267 ) ) ;
#65462=CARTESIAN_POINT ( 'NONE',  ( 17.74745361342931105, -281.6380170796243192, -324.0888299054577146 ) ) ;
#65463=CARTESIAN_POINT ( 'NONE',  ( 26.06522289078438348, -274.3255459448911893, -226.8305931864368574 ) ) ;
#65464=CARTESIAN_POINT ( 'NONE',  ( -110.9255369692004081, -282.4820745524079371, -281.9501052623288047 ) ) ;
#65465=CARTESIAN_POINT ( 'NONE',  ( -39.54351107313486580, -278.4248479933576732, -194.1800173669438436 ) ) ;
#65466=CARTESIAN_POINT ( 'NONE',  ( -87.68424627207404853, -277.3507448703946352, -214.5430521636019989 ) ) ;
#65468=CARTESIAN_POINT ( 'NONE',  ( -73.07208807262840367, -296.2527589669163604, -206.1382026333387216 ) ) ;
#65469=CARTESIAN_POINT ( 'NONE',  ( 35.00224187855551605, -277.8072619752724677, -290.1918125183523216 ) ) ;
#65471=CARTESIAN_POINT ( 'NONE',  ( -17.04487854568082739, -290.3330541484819491, -197.7908359538226080 ) ) ;
#65472=CARTESIAN_POINT ( 'NONE',  ( -113.6661420330862597, -290.6843165575915577, -259.7933605849357264 ) ) ;
#65473=CARTESIAN_POINT ( 'NONE',  ( -31.43026629616741019, -276.1267746477807350, -195.4142928862090969 ) ) ;
#65474=CARTESIAN_POINT ( 'NONE',  ( -50.24562860623797889, -295.8868865773580410, -196.6487238169881664 ) ) ;
#65475=CARTESIAN_POINT ( 'NONE',  ( -105.2845240311445565, -284.2149525763747988, -234.3594596461950630 ) ) ;
#65476=DIRECTION ( 'NONE',  ( 0.000000000000000000, -1.000000000000000000, 0.000000000000000000 ) ) ;
#65477=CARTESIAN_POINT ( 'NONE',  ( -89.27099874892783760, -281.7823620416045856, -324.5464073047963893 ) ) ;
#65480=CARTESIAN_POINT ( 'NONE',  ( -30.75614646379407802, -290.9321736974778219, -197.2600852417377268 ) ) ;
#65481=CARTESIAN_POINT ( 'NONE',  ( -98.35791083786813260, -283.2713305277754330, -228.0552393574312759 ) ) ;
#65484=CARTESIAN_POINT ( 'NONE',  ( 34.24848929151041688, -291.8403679683247560, -292.7183411551075096 ) ) ;
#65485=CARTESIAN_POINT ( 'NONE',  ( -96.64590069198710864, -282.3819847786404580, -318.3995661443665881 ) ) ;
#65486=CARTESIAN_POINT ( 'NONE',  ( -24.16698785917438386, -278.4813948826387673, -343.0276467161061760 ) ) ;
#65487=CARTESIAN_POINT ( 'NONE',  ( -69.63947779557744866, -286.8414734742384553, -200.8855970613653881 ) ) ;
#65488=CARTESIAN_POINT ( 'NONE',  ( -103.4854645873572423, -284.9706639195849220, -239.3543580956023789 ) ) ;
#65489=CARTESIAN_POINT ( 'NONE',  ( -41.87489294667201278, -278.5356331447423486, -343.8232890791103387 ) ) ;
#65490=CARTESIAN_POINT ( 'NONE',  ( -104.5945117932865855, -279.7410652754268199, -241.5572805714275546 ) ) ;
#65491=CARTESIAN_POINT ( 'NONE',  ( -88.54005977374177405, -287.3348173336079867, -215.4841763608947929 ) ) ;
#65492=EDGE_LOOP ( 'NONE', ( #57174, #68774 ) ) ;
#65493=CARTESIAN_POINT ( 'NONE',  ( -70.80979128418196922, -295.3147306903626941, -339.7217663970918693 ) ) ;
#65494=CARTESIAN_POINT ( 'NONE',  ( -31.72293498328045658, -290.9609173104047386, -344.8459143688191375 ) ) ;
#65496=CARTESIAN_POINT ( 'NONE',  ( 13.79469577742117714, -283.1948066931273615, -206.1857440867352693 ) ) ;
#65498=CARTESIAN_POINT ( 'NONE',  ( 23.37902115964356753, -292.5718400968868877, -316.3984335418881528 ) ) ;
#65499=CARTESIAN_POINT ( 'NONE',  ( 34.05552348880730307, -288.8330223627122564, -252.0579997104457846 ) ) ;
#65500=CARTESIAN_POINT ( 'NONE',  ( -92.06089399243730043, -281.0171072878628138, -220.5235434321706975 ) ) ;
#65501=CARTESIAN_POINT ( 'NONE',  ( 25.37852856722543748, -289.5596237458603923, -314.0957705816539374 ) ) ;
#65502=CARTESIAN_POINT ( 'NONE',  ( -99.16696148391430654, -285.9759625279380089, -312.9090712521626756 ) ) ;
#65503=CARTESIAN_POINT ( 'NONE',  ( -112.0864308805788454, -278.9508717504500623, -251.8076854871989951 ) ) ;
#65505=CARTESIAN_POINT ( 'NONE',  ( -2.650793769281881040, -292.6768713481646955, -337.4867853306007532 ) ) ;
#65506=CARTESIAN_POINT ( 'NONE',  ( -3.655691844096808918, -280.3177541915674738, -201.1060561584997686 ) ) ;
#65508=CARTESIAN_POINT ( 'NONE',  ( -65.05148502367389085, -275.5466795367907480, -201.4777244248728607 ) ) ;
#65510=CARTESIAN_POINT ( 'NONE',  ( -37.37352853689063892, -288.5519495502701943, -195.3611179825600175 ) ) ;
#65511=CARTESIAN_POINT ( 'NONE',  ( -65.82628503182380086, -271.9244892412024797, -199.9013952259350617 ) ) ;
#65514=CARTESIAN_POINT ( 'NONE',  ( -105.5695062337035495, -278.4102139373451337, -244.0860417251003582 ) ) ;
#65516=CARTESIAN_POINT ( 'NONE',  ( -4.152925742680994681, -277.8293433113927335, -339.4154884680469308 ) ) ;
#65517=CARTESIAN_POINT ( 'NONE',  ( -110.8348508120440101, -273.8671145409825840, -270.3778243577502280 ) ) ;
#65518=CARTESIAN_POINT ( 'NONE',  ( -85.96262405029688125, -282.7659978014171429, -329.7650401529969599 ) ) ;
#65519=CARTESIAN_POINT ( 'NONE',  ( -111.1310151358370888, -292.2293141695091094, -276.7392357874032314 ) ) ;
#65520=CARTESIAN_POINT ( 'NONE',  ( -9.445442236418003290, -299.9155321296868237, -194.0473822636144519 ) ) ;
#65522=CARTESIAN_POINT ( 'NONE',  ( -60.04512324328197082, -298.9694991932984180, -197.1446637508538515 ) ) ;
#65523=CARTESIAN_POINT ( 'NONE',  ( 4.871037225636397849, -296.4805289426475383, -332.1520010429561580 ) ) ;
#65524=CARTESIAN_POINT ( 'NONE',  ( -108.7425469832865872, -282.2623234403394576, -292.7653027514992345 ) ) ;
#65526=CARTESIAN_POINT ( 'NONE',  ( -105.8801740222697561, -270.9623925700839209, -240.6612547418662871 ) ) ;
#65527=CARTESIAN_POINT ( 'NONE',  ( 34.09706668135849839, -288.8135444252168327, -243.8480455293226896 ) ) ;
#65528=ADVANCED_FACE ( 'NONE', ( #51086, #15112 ), #6626, .T. ) ;
#65529=CARTESIAN_POINT ( 'NONE',  ( -10.62420498176592965, -287.6157347416850030, -338.6826924085395945 ) ) ;
#65530=CARTESIAN_POINT ( 'NONE',  ( -110.9628874742100777, -271.9671495687064748, -296.3246994010440858 ) ) ;
#65531=EDGE_LOOP ( 'NONE', ( #47544, #80171, #58562, #66012 ) ) ;
#65532=CARTESIAN_POINT ( 'NONE',  ( -113.5265521581347201, -289.0446614328807868, -276.8850786413128731 ) ) ;
#65533=CARTESIAN_POINT ( 'NONE',  ( 16.02351505426820566, -287.9362158221861705, -320.2772619269998131 ) ) ;
#65534=ORIENTED_EDGE ( 'NONE', *, *, #28465, .T. ) ;
#65535=CARTESIAN_POINT ( 'NONE',  ( -69.67509314950392252, -286.7160894653333685, -200.8051369070755641 ) ) ;
#65537=CARTESIAN_POINT ( 'NONE',  ( -64.33701090352067808, -277.7475424969254050, -338.2627374946621330 ) ) ;
#65539=CARTESIAN_POINT ( 'NONE',  ( 36.79421480341117956, -292.7192364340471613, -289.9916714093535575 ) ) ;
#65540=CARTESIAN_POINT ( 'NONE',  ( -30.21606924908947533, -283.6156446163547571, -346.9283314038112280 ) ) ;
#65541=CARTESIAN_POINT ( 'NONE',  ( 37.46966477689971242, -283.2619751327841300, -285.3933312492559935 ) ) ;
#65542=CARTESIAN_POINT ( 'NONE',  ( -52.90918733402959617, -283.5795723328850499, -345.8039067124552730 ) ) ;
#65543=CARTESIAN_POINT ( 'NONE',  ( 27.79833626442015415, -281.4361868750625604, -237.2510877576574160 ) ) ;
#65544=CARTESIAN_POINT ( 'NONE',  ( 121.9602794296661017, 149.5214840255910360, -263.6741255141749889 ) ) ;
#65545=CARTESIAN_POINT ( 'NONE',  ( -111.3001811514157851, -280.4054939237981330, -281.7703910497300512 ) ) ;
#65546=CARTESIAN_POINT ( 'NONE',  ( -108.4282835402909200, -261.3898650898953520, -317.1797982494042003 ) ) ;
#65547=CARTESIAN_POINT ( 'NONE',  ( -108.9999068415822450, -263.8798383989249601, -305.4964869628947781 ) ) ;
#65549=CARTESIAN_POINT ( 'NONE',  ( -35.37576289747776315, -273.2745857515132570, -197.2135263685501627 ) ) ;
#65550=CARTESIAN_POINT ( 'NONE',  ( -16.52955750363717868, -294.2980092150471023, -344.4864180480755635 ) ) ;
#65551=CARTESIAN_POINT ( 'NONE',  ( 139.3042675125565211, 178.0593506817157561, -238.4361927324221995 ) ) ;
#65552=CARTESIAN_POINT ( 'NONE',  ( -80.95542691221804432, -272.1587295010256184, -207.4388264342572654 ) ) ;
#65553=CARTESIAN_POINT ( 'NONE',  ( -100.9674855778340685, -298.9311831010950300, -232.0168203863419478 ) ) ;
#65554=CARTESIAN_POINT ( 'NONE',  ( 30.94959958044641724, -289.2298844993276248, -297.6561756056091781 ) ) ;
#65556=CARTESIAN_POINT ( 'NONE',  ( -61.50609399691204260, -296.2996758059447302, -343.2788974716046368 ) ) ;
#65557=CARTESIAN_POINT ( 'NONE',  ( -38.63227807983282958, -286.5279199974649487, -197.2984865787412332 ) ) ;
#65558=CARTESIAN_POINT ( 'NONE',  ( -49.65599822687256193, -272.8191005767642423, -194.6117532226535616 ) ) ;
#65560=CARTESIAN_POINT ( 'NONE',  ( 37.90169481907362581, -294.1589728779382540, -254.7213592204973338 ) ) ;
#65561=CARTESIAN_POINT ( 'NONE',  ( -0.8385869307530524619, -293.0160264751180534, -202.6333568335425070 ) ) ;
#65562=CARTESIAN_POINT ( 'NONE',  ( -64.07358651758011092, -291.8601918360130298, -202.4181636152756880 ) ) ;
#65563=ORIENTED_EDGE ( 'NONE', *, *, #2379, .F. ) ;
#65564=CARTESIAN_POINT ( 'NONE',  ( -27.21419690957961279, -276.0999279833812352, -195.4304681298480375 ) ) ;
#65565=CARTESIAN_POINT ( 'NONE',  ( 39.15877469630972030, -274.2857222915546913, -265.4804497280269970 ) ) ;
#65567=CARTESIAN_POINT ( 'NONE',  ( -99.60365762841171033, -277.4593997588095817, -315.5828097142248225 ) ) ;
#65569=CARTESIAN_POINT ( 'NONE',  ( -3.722251669737950408, -272.9032473839519071, -204.6493414318743476 ) ) ;
#65570=CARTESIAN_POINT ( 'NONE',  ( -51.63513270364259000, -274.9448179925313980, -198.4069245620116817 ) ) ;
#65571=CARTESIAN_POINT ( 'NONE',  ( 30.38786864103631657, -276.1196300856387325, -242.3691887509122012 ) ) ;
#65572=CARTESIAN_POINT ( 'NONE',  ( -101.8704918431633786, -274.8441914698143478, -230.2361998846719757 ) ) ;
#65573=CARTESIAN_POINT ( 'NONE',  ( -3.487147892860260168, -274.6276798500598488, -337.6976617855184486 ) ) ;
#65574=CARTESIAN_POINT ( 'NONE',  ( -94.01631526056149823, -296.5506896284615550, -316.5530822314275383 ) ) ;
#65575=CARTESIAN_POINT ( 'NONE',  ( 31.12717615511658664, -292.4863139314028331, -297.4705808300105332 ) ) ;
#65577=CARTESIAN_POINT ( 'NONE',  ( -106.2874478220169863, -278.6039259086215907, -304.6278647257012722 ) ) ;
#65578=CARTESIAN_POINT ( 'NONE',  ( -2.915533270563619883, -274.6872931473909603, -205.9884604327900774 ) ) ;
#65579=CARTESIAN_POINT ( 'NONE',  ( -111.8754825022579951, -283.4542770260279667, -253.0980487261579981 ) ) ;
#65580=CARTESIAN_POINT ( 'NONE',  ( -94.17814276327253253, -297.8715440682574922, -319.5510276953405651 ) ) ;
#65582=AXIS2_PLACEMENT_3D ( 'NONE', #92552, #42842, #71278 ) ;
#65583=CARTESIAN_POINT ( 'NONE',  ( -41.32151313304918006, -285.1979647738228323, -197.2954412939511144 ) ) ;
#65584=CARTESIAN_POINT ( 'NONE',  ( -87.80255211493745549, -276.0089338905548857, -324.5060755362359828 ) ) ;
#65585=CARTESIAN_POINT ( 'NONE',  ( -94.07177930449284986, -276.4675461529768086, -317.2538134764875508 ) ) ;
#65586=CARTESIAN_POINT ( 'NONE',  ( -112.3502763745730562, -286.5198263715149096, -272.8915676756419657 ) ) ;
#65587=CARTESIAN_POINT ( 'NONE',  ( 23.37220969433365525, -276.1864920688550455, -229.0959857785408360 ) ) ;
#65590=CARTESIAN_POINT ( 'NONE',  ( 33.43356009749853541, -274.3156399060009107, -298.7398347481271230 ) ) ;
#65591=AXIS2_PLACEMENT_3D ( 'NONE', #27457, #71020, #64422 ) ;
#65592=CARTESIAN_POINT ( 'NONE',  ( -50.64088620623854098, -281.8828257183184292, -196.3803091640184562 ) ) ;
#65593=CARTESIAN_POINT ( 'NONE',  ( 38.26201954786014880, -289.4868819838978311, -271.5046274318437440 ) ) ;
#65595=CARTESIAN_POINT ( 'NONE',  ( 34.91680843867518291, -291.8126063833635726, -290.6402828075584353 ) ) ;
#65596=CARTESIAN_POINT ( 'NONE',  ( 82.17160520760587872, -297.7678833447943703, -196.2839431741979297 ) ) ;
#65597=CARTESIAN_POINT ( 'NONE',  ( -102.4596836479148863, -271.6988677413764321, -236.1790809474917125 ) ) ;
#65598=CARTESIAN_POINT ( 'NONE',  ( -93.47523585989389971, -289.3724734215381318, -221.7824019793234527 ) ) ;
#65599=CARTESIAN_POINT ( 'NONE',  ( 30.52007695399996479, -26.23604800832216100, -343.5755449821854768 ) ) ;
#65600=CARTESIAN_POINT ( 'NONE',  ( -70.10895070716225064, -295.6202805390466324, -202.8977357441297613 ) ) ;
#65601=CARTESIAN_POINT ( 'NONE',  ( -8.513175731833138471, -287.1614981346177160, -341.0266796032209413 ) ) ;
#65602=CARTESIAN_POINT ( 'NONE',  ( -112.8105724428530010, -282.9042424062359942, -261.5054235241709648 ) ) ;
#65604=CARTESIAN_POINT ( 'NONE',  ( -83.14742077496897821, -285.1184776164806181, -328.0217259743778868 ) ) ;
#65605=CARTESIAN_POINT ( 'NONE',  ( -97.65969248434043948, -284.7788278585090325, -311.8540038671407615 ) ) ;
#65606=CARTESIAN_POINT ( 'NONE',  ( -51.35419568960561776, -291.2103653891529689, -344.4020307813381123 ) ) ;
#65607=CARTESIAN_POINT ( 'NONE',  ( -63.55388432643461982, -274.0529384340632078, -197.9824906741909842 ) ) ;
#65609=CARTESIAN_POINT ( 'NONE',  ( 30.38564262801431681, -286.0720870260548736, -303.9801053340400472 ) ) ;
#65610=CARTESIAN_POINT ( 'NONE',  ( 29.94753258409132712, -275.0656987043681738, -232.8194162944809307 ) ) ;
#65611=CARTESIAN_POINT ( 'NONE',  ( 35.68180583284402729, -295.7324524997122239, -285.8955450662704152 ) ) ;
#65613=CARTESIAN_POINT ( 'NONE',  ( -69.85430415644619018, -297.9805209788416391, -337.9475929042657754 ) ) ;
#65614=CARTESIAN_POINT ( 'NONE',  ( -40.27066669121460052, -281.7745612761715392, -343.7958824602116579 ) ) ;
#65615=CARTESIAN_POINT ( 'NONE',  ( -93.84978376405879885, -275.8649272231995155, -319.9278902430459652 ) ) ;
#65616=CARTESIAN_POINT ( 'NONE',  ( -46.77591700506830819, -272.4143134296629114, -194.6398970231161627 ) ) ;
#65617=CARTESIAN_POINT ( 'NONE',  ( -6.240783130062105499, -275.9809884557118380, -336.5309750321059141 ) ) ;
#65619=CARTESIAN_POINT ( 'NONE',  ( 2.600182152513579759, -294.1181409809346405, -208.3704448016505637 ) ) ;
#65621=CARTESIAN_POINT ( 'NONE',  ( 34.30024907722243910, -294.6939803633845258, -285.6147210171870938 ) ) ;
#65622=CARTESIAN_POINT ( 'NONE',  ( 34.88961699931628857, -294.6589912247051188, -245.2763189657629823 ) ) ;
#65623=CARTESIAN_POINT ( 'NONE',  ( 19.99791316113373085, -294.1767997048375491, -219.6908910885088346 ) ) ;
#65624=CARTESIAN_POINT ( 'NONE',  ( -107.4587765877218288, -296.6541364877508045, -250.0486687637107934 ) ) ;
#65625=CARTESIAN_POINT ( 'NONE',  ( -111.5996612287716090, -292.4160058654288150, -280.9770965847881712 ) ) ;
#65626=CARTESIAN_POINT ( 'NONE',  ( -96.26894314102001715, -284.0512335491926024, -319.9454166209545178 ) ) ;
#65627=CARTESIAN_POINT ( 'NONE',  ( -93.21803652644112503, -271.3992645476581629, -219.1742014041453785 ) ) ;
#65628=CARTESIAN_POINT ( 'NONE',  ( -20.98189734052662558, -286.0898370103569164, -195.1191293243878988 ) ) ;
#65629=CARTESIAN_POINT ( 'NONE',  ( -26.76406421823233472, -278.8968461953814426, -344.2526629606987854 ) ) ;
#65630=CARTESIAN_POINT ( 'NONE',  ( -105.9305712482647834, -283.6940511114416950, -244.2326418962472871 ) ) ;
#65631=CARTESIAN_POINT ( 'NONE',  ( 23.92640212349585127, -284.9640712534156819, -227.0813618578237367 ) ) ;
#65632=CARTESIAN_POINT ( 'NONE',  ( -90.17949863009447142, -277.4547054888250273, -215.9881621528031701 ) ) ;
#65633=CARTESIAN_POINT ( 'NONE',  ( -117.0946091816712453, -269.6096274233381109, -270.3236525939013859 ) ) ;
#65634=CARTESIAN_POINT ( 'NONE',  ( 30.73134748356642376, -283.2123812505230376, -305.4904348895843214 ) ) ;
#65635=AXIS2_PLACEMENT_3D ( 'NONE', #41835, #26715, #62728 ) ;
#65636=CARTESIAN_POINT ( 'NONE',  ( 10.07317217267784137, -287.4757265666959256, -330.7996713298073814 ) ) ;
#65637=CARTESIAN_POINT ( 'NONE',  ( -94.59609192810681577, -279.4646343958065700, -320.6440677386422635 ) ) ;
#65638=CARTESIAN_POINT ( 'NONE',  ( -2.931808993251968865, -277.9222129484760444, -338.7076699259418433 ) ) ;
#65639=CARTESIAN_POINT ( 'NONE',  ( -68.52136485102623453, -279.4639430213114224, -204.3548416726315509 ) ) ;
#65640=CARTESIAN_POINT ( 'NONE',  ( 34.46282722726831338, -293.1982532621263999, -242.4089174557115598 ) ) ;
#65641=CARTESIAN_POINT ( 'NONE',  ( 4.516562378373683018, -286.5048284922152675, -332.2274174111881280 ) ) ;
#65642=CARTESIAN_POINT ( 'NONE',  ( -97.72692606006464189, -292.7791532713339961, -223.8634983215192165 ) ) ;
#65643=CARTESIAN_POINT ( 'NONE',  ( -18.15277336290058585, -293.7192567396938898, -341.1142886700226313 ) ) ;
#65644=CARTESIAN_POINT ( 'NONE',  ( 22.94804982942261873, -293.7930158145457540, -311.6470271200916500 ) ) ;
#65645=CARTESIAN_POINT ( 'NONE',  ( -111.3381887744287013, -291.8857677029655520, -250.1615096632381778 ) ) ;
#65646=CARTESIAN_POINT ( 'NONE',  ( 29.41092191300931802, -282.6057562661483189, -300.2844335558414173 ) ) ;
#65648=CARTESIAN_POINT ( 'NONE',  ( -114.1059607011668362, -271.6469132745270940, -267.4904571022046866 ) ) ;
#65649=CARTESIAN_POINT ( 'NONE',  ( -43.16628952759693050, -289.7752909140342013, -347.0382784994224039 ) ) ;
#65650=CARTESIAN_POINT ( 'NONE',  ( -63.50801472316615559, -281.5291653128440430, -341.4640677133127724 ) ) ;
#65651=CARTESIAN_POINT ( 'NONE',  ( -41.75510213338536403, -289.4395742089017745, -347.2265725225928463 ) ) ;
#65652=CARTESIAN_POINT ( 'NONE',  ( -46.73179300374368239, -286.2630749785448643, -197.8954559741196988 ) ) ;
#65653=CARTESIAN_POINT ( 'NONE',  ( 104.2209783822911646, -299.5541904835127980, -195.3611179825600175 ) ) ;
#65655=CARTESIAN_POINT ( 'NONE',  ( 101.4506851708696473, 116.4004253888254112, -281.2237119222594970 ) ) ;
#65656=CARTESIAN_POINT ( 'NONE',  ( -109.9537836488778026, -268.4403653933277383, -295.2708550661919276 ) ) ;
#65657=CARTESIAN_POINT ( 'NONE',  ( -94.05924625524917815, -278.4020502465177174, -224.1472489729320614 ) ) ;
#65658=CARTESIAN_POINT ( 'NONE',  ( -19.44584356988162810, -279.2079903894094741, -199.2173638768322235 ) ) ;
#65659=CARTESIAN_POINT ( 'NONE',  ( -46.87417256749950667, -273.6009629694686396, -193.9747562373963490 ) ) ;
#65660=CARTESIAN_POINT ( 'NONE',  ( 198.3562286197148410, 281.9606030181009828, -110.7138469406835100 ) ) ;
#65661=CARTESIAN_POINT ( 'NONE',  ( -97.22372735001258093, -277.7669456291655479, -222.8979837474010139 ) ) ;
#65663=CARTESIAN_POINT ( 'NONE',  ( -103.2347835030742402, -282.1036022958002150, -305.5418156893044284 ) ) ;
#65664=CARTESIAN_POINT ( 'NONE',  ( -39.06212939791685557, -296.8335992799869132, -346.3283091877803486 ) ) ;
#65665=CARTESIAN_POINT ( 'NONE',  ( -25.40520933008716753, -292.7006154623310294, -198.2297198930030504 ) ) ;
#65666=CARTESIAN_POINT ( 'NONE',  ( -96.96846295032291607, -288.6401845323081830, -313.3249706284229319 ) ) ;
#65667=CARTESIAN_POINT ( 'NONE',  ( -36.54771265828082960, -298.5541877098402210, -193.4225916368854996 ) ) ;
#65668=CARTESIAN_POINT ( 'NONE',  ( -110.2124125022334056, -296.7761210569072432, -266.0183904329023790 ) ) ;
#65673=CARTESIAN_POINT ( 'NONE',  ( -109.1882311765221658, -280.7741451873852156, -246.7985140577095819 ) ) ;
#65675=CARTESIAN_POINT ( 'NONE',  ( -32.95821086214761664, -281.1883489703806163, -197.1831766622930218 ) ) ;
#65676=CARTESIAN_POINT ( 'NONE',  ( -102.7223172990467219, -279.7999245629074494, -309.1856785222297503 ) ) ;
#65677=CARTESIAN_POINT ( 'NONE',  ( 14.08138906443866389, -281.3674728372805021, -322.5772519283208908 ) ) ;
#65678=CARTESIAN_POINT ( 'NONE',  ( 7.770473463442780115, -273.1610053400829088, -212.0893448470239377 ) ) ;
#65680=CARTESIAN_POINT ( 'NONE',  ( 31.10181793048083776, -275.9042495949026943, -235.4377210147539188 ) ) ;
#65683=CARTESIAN_POINT ( 'NONE',  ( 21.18132166857535736, -276.9069961144561489, -223.4360010145438764 ) ) ;
#65684=CARTESIAN_POINT ( 'NONE',  ( -105.8254036949802810, -276.6866149929853691, -304.3710524893692764 ) ) ;
#65687=CARTESIAN_POINT ( 'NONE',  ( 8.234473884295582025, -284.4119733970817947, -330.3712768076471207 ) ) ;
#65688=CARTESIAN_POINT ( 'NONE',  ( -94.41045300740755408, -290.3951056187565314, -224.5617513141136499 ) ) ;
#65689=CARTESIAN_POINT ( 'NONE',  ( 20.21597755516480532, -286.2083622571286696, -219.2881259666707194 ) ) ;
#65690=CARTESIAN_POINT ( 'NONE',  ( -106.1643664325362977, -282.4311266026384715, -297.7296655066767812 ) ) ;
#65691=CARTESIAN_POINT ( 'NONE',  ( -64.28789304075455391, -281.9855355132146997, -338.8394182314698355 ) ) ;
#65692=CARTESIAN_POINT ( 'NONE',  ( 36.42649006824807856, -285.4980268198166868, -260.0053142912898920 ) ) ;
#65693=CARTESIAN_POINT ( 'NONE',  ( 36.08423256897204823, -282.7335852743458418, -268.5585956335388005 ) ) ;
#65694=CARTESIAN_POINT ( 'NONE',  ( -70.49517678076114180, -271.6148902126982421, -203.0866975912457519 ) ) ;
#65695=CARTESIAN_POINT ( 'NONE',  ( -78.07740889624230363, -283.9140962488267519, -205.9635835141338873 ) ) ;
#65696=CARTESIAN_POINT ( 'NONE',  ( -50.10153223322036098, -297.2150176968947335, -344.3202717463917679 ) ) ;
#65697=CARTESIAN_POINT ( 'NONE',  ( -109.8565215871018097, -279.6327864380735377, -259.7614434809553927 ) ) ;
#65698=CARTESIAN_POINT ( 'NONE',  ( -97.88314763658974016, -287.1595758941229519, -225.7247776145287901 ) ) ;
#65700=EDGE_CURVE ( 'NONE', #60383, #34864, #53448, .T. ) ;
#65701=ADVANCED_FACE ( 'NONE', ( #43066, #56835 ), #63471, .T. ) ;
#65703=CARTESIAN_POINT ( 'NONE',  ( 36.66523498722360586, -295.6665438404938300, -285.6021073289408037 ) ) ;
#65704=CARTESIAN_POINT ( 'NONE',  ( -109.5367807850850994, -276.8139732431921516, -249.9943505465527380 ) ) ;
#65705=CARTESIAN_POINT ( 'NONE',  ( 5.458883239541190591, -287.6857301087448491, -334.1754493158779269 ) ) ;
#65706=CARTESIAN_POINT ( 'NONE',  ( 20.82589295685690800, -291.3185550414207228, -224.9207061888733961 ) ) ;
#65707=CARTESIAN_POINT ( 'NONE',  ( -110.1076733507587875, -277.3767244782780494, -259.6956278307153525 ) ) ;
#65708=CARTESIAN_POINT ( 'NONE',  ( -109.0222737768553714, -294.9430807871445381, -251.0051783274368518 ) ) ;
#65709=CARTESIAN_POINT ( 'NONE',  ( -28.06056005679196730, -293.4874622176997150, -197.4052683278934808 ) ) ;
#65712=CARTESIAN_POINT ( 'NONE',  ( -96.87874999216938932, -294.3865439936605526, -318.1106985191667036 ) ) ;
#65713=CARTESIAN_POINT ( 'NONE',  ( 35.07305991042505866, -289.3388423106831624, -284.6582934687115198 ) ) ;
#65714=CARTESIAN_POINT ( 'NONE',  ( -105.6130552401944698, -288.3565481772901080, -303.8423876487195230 ) ) ;
#65715=CARTESIAN_POINT ( 'NONE',  ( -82.89692537335099587, -291.1148297998149133, -328.1546848241031284 ) ) ;
#65717=CARTESIAN_POINT ( 'NONE',  ( -61.29825842609412945, -290.1742260355367762, -339.4891516687136459 ) ) ;
#65718=DIRECTION ( 'NONE',  ( 0.000000000000000000, 0.000000000000000000, -1.000000000000000000 ) ) ;
#65719=CARTESIAN_POINT ( 'NONE',  ( -45.96574628048999500, -290.3641362977431868, -346.5298986650830102 ) ) ;
#65720=CARTESIAN_POINT ( 'NONE',  ( -3.114213563330051393, -278.5220781646007708, -203.2133581906317659 ) ) ;
#65722=CARTESIAN_POINT ( 'NONE',  ( -100.2341611294646242, -279.4729289279294449, -225.9732520647272622 ) ) ;
#65723=CARTESIAN_POINT ( 'NONE',  ( 27.83571258969580597, -280.6812965225213929, -229.3020978850011034 ) ) ;
#65724=CARTESIAN_POINT ( 'NONE',  ( 1.218207418715790968, -284.5664680352350047, -205.9722292622062128 ) ) ;
#65725=CARTESIAN_POINT ( 'NONE',  ( -111.9369532652702759, -274.5219144271438836, -270.3861977745045237 ) ) ;
#65726=CARTESIAN_POINT ( 'NONE',  ( -75.11421913820873897, -277.6831422793591173, -206.3950612263149935 ) ) ;
#65727=CARTESIAN_POINT ( 'NONE',  ( -108.3398298335461192, -282.2393248531168410, -294.5327175635376875 ) ) ;
#65728=CARTESIAN_POINT ( 'NONE',  ( -110.6395987583250218, -271.3322271344074466, -283.6871842494841758 ) ) ;
#65729=CARTESIAN_POINT ( 'NONE',  ( -88.75933643169038589, -276.2385731889982594, -326.7431579257748240 ) ) ;
#65731=CARTESIAN_POINT ( 'NONE',  ( -99.54585721581733537, -282.8743313558071009, -315.3067171856280311 ) ) ;
#65732=CARTESIAN_POINT ( 'NONE',  ( -62.09392073361606634, -274.5247187052497679, -201.5139735104079364 ) ) ;
#65733=CARTESIAN_POINT ( 'NONE',  ( -94.06769170125781443, -292.8149470727479979, -223.1333081359151151 ) ) ;
#65734=CARTESIAN_POINT ( 'NONE',  ( -106.3191677418332262, -274.4020936240484048, -237.4868841074855936 ) ) ;
#65735=CARTESIAN_POINT ( 'NONE',  ( 33.53072730108748800, -274.9869032304191592, -252.7774176564259108 ) ) ;
#65736=CARTESIAN_POINT ( 'NONE',  ( -71.82837730128250087, -297.5080765006804882, -336.9763073938436264 ) ) ;
#65737=CARTESIAN_POINT ( 'NONE',  ( -3.058825391129794458, -288.7784952172309545, -339.3227154887462689 ) ) ;
#65739=CARTESIAN_POINT ( 'NONE',  ( 7.707977552399481347, -278.7411913623584496, -209.6343727137316648 ) ) ;
#65741=CARTESIAN_POINT ( 'NONE',  ( -44.89493376068840291, -291.7924912679493445, -193.6795543714625012 ) ) ;
#65742=CARTESIAN_POINT ( 'NONE',  ( -80.55598004052031058, -288.7127549137894107, -329.5506581157301866 ) ) ;
#65743=CARTESIAN_POINT ( 'NONE',  ( 0.7316197033791036475, -292.5442274642832103, -334.9786308242219661 ) ) ;
#65746=CARTESIAN_POINT ( 'NONE',  ( -97.40306850759695578, -289.4804311648698558, -311.9838270009958023 ) ) ;
#65748=CARTESIAN_POINT ( 'NONE',  ( -10.08874079242265864, -287.3405109877057271, -198.5403222640659351 ) ) ;
#65749=CARTESIAN_POINT ( 'NONE',  ( -53.28691492658256834, -291.7662352645559167, -340.3683826091709079 ) ) ;
#65750=CARTESIAN_POINT ( 'NONE',  ( -3.343807019167917005, -293.6730350296325582, -339.2012783089644472 ) ) ;
#65751=CARTESIAN_POINT ( 'NONE',  ( -37.29761397685438595, -284.3667421951370216, -346.8809382987477647 ) ) ;
#65752=CARTESIAN_POINT ( 'NONE',  ( -107.3925195957829999, -284.1131946362799567, -290.9455367621443429 ) ) ;
#65753=CARTESIAN_POINT ( 'NONE',  ( 36.19254153326932766, -276.8832591651515713, -271.5765208383338063 ) ) ;
#65754=CARTESIAN_POINT ( 'NONE',  ( 7.020668168854167668, -292.4653329778913644, -330.4574020605629698 ) ) ;
#65756=CARTESIAN_POINT ( 'NONE',  ( 34.76645693901235035, -274.1673948292336149, -256.6664405452803521 ) ) ;
#65758=CARTESIAN_POINT ( 'NONE',  ( 202.9738562182569694, 296.4636489450776367, -53.99999999999997868 ) ) ;
#65759=CARTESIAN_POINT ( 'NONE',  ( 6.598450208492826263, -294.1397526369988213, -333.6321373547042413 ) ) ;
#65760=CARTESIAN_POINT ( 'NONE',  ( 21.46346364243232685, -288.8418198304104862, -224.7182991022280021 ) ) ;
#65761=CARTESIAN_POINT ( 'NONE',  ( -114.0566262001358808, -297.6052779302710292, -272.4750473502695058 ) ) ;
#65762=CARTESIAN_POINT ( 'NONE',  ( 28.89882605107830926, -287.7866190791410759, -239.4404879867815623 ) ) ;
#65763=CARTESIAN_POINT ( 'NONE',  ( -75.23052950073038403, -276.6031842415533788, -337.1238083256711207 ) ) ;
#65764=CARTESIAN_POINT ( 'NONE',  ( 17.49468440942154146, -294.9453288962300803, -324.3468227384097986 ) ) ;
#65765=CARTESIAN_POINT ( 'NONE',  ( -20.78970478231500607, -286.9816053300080512, -344.3495844638194967 ) ) ;
#65766=CARTESIAN_POINT ( 'NONE',  ( 17.54944698480496612, -294.6272481452900251, -324.4064325299128200 ) ) ;
#65767=CARTESIAN_POINT ( 'NONE',  ( -64.08330407746979063, -292.0267660864091113, -202.3992612715831854 ) ) ;
#65770=CARTESIAN_POINT ( 'NONE',  ( 197.1939414079469941, 281.6276418468785323, -110.3312364698208228 ) ) ;
#65771=CARTESIAN_POINT ( 'NONE',  ( 38.88388837170287360, -289.0152164241742980, -265.8400043962846553 ) ) ;
#65772=CARTESIAN_POINT ( 'NONE',  ( -115.3288506153726871, -282.2666405000203440, -252.5284128619063608 ) ) ;
#65774=CARTESIAN_POINT ( 'NONE',  ( -42.41503485917646543, -279.3383343500467504, -193.6305891080372987 ) ) ;
#65775=CARTESIAN_POINT ( 'NONE',  ( 20.79197628991754954, -284.2028694440267600, -317.5035491278106292 ) ) ;
#65776=CARTESIAN_POINT ( 'NONE',  ( -82.90982830526120040, -284.0175113988842099, -208.9587649944826637 ) ) ;
#65777=CARTESIAN_POINT ( 'NONE',  ( 23.92137006911448793, -286.2098281693962463, -312.6701039471620902 ) ) ;
#65778=CARTESIAN_POINT ( 'NONE',  ( -18.87435577062038305, -276.1477190557915833, -196.8272996567008022 ) ) ;
#65779=CARTESIAN_POINT ( 'NONE',  ( -37.82921519546573563, -298.5382312439015209, -197.3012057807513315 ) ) ;
#65780=CARTESIAN_POINT ( 'NONE',  ( 1.818531145371408364, -293.2015125376300944, -332.6123761224383202 ) ) ;
#65781=CARTESIAN_POINT ( 'NONE',  ( -56.53923668610484299, -280.4625498478460486, -195.8429940424889537 ) ) ;
#65782=CARTESIAN_POINT ( 'NONE',  ( 25.37557032388277634, -276.0657500860480695, -307.7180984153411600 ) ) ;
#65783=CARTESIAN_POINT ( 'NONE',  ( -110.4939669181725606, -277.8971905212325169, -270.6301615191002838 ) ) ;
#65784=CARTESIAN_POINT ( 'NONE',  ( -55.27472808253266834, -274.9063457531331665, -195.7963875984286517 ) ) ;
#65785=CARTESIAN_POINT ( 'NONE',  ( -2.876395262564094057, -275.5277549784264011, -338.8858466805365310 ) ) ;
#65786=CARTESIAN_POINT ( 'NONE',  ( 173.6393091185710489, 243.4999469643735210, -179.6212980619924622 ) ) ;
#65787=CARTESIAN_POINT ( 'NONE',  ( 16.76155902123706198, -274.2824089246178687, -322.3749276737877949 ) ) ;
#65788=CARTESIAN_POINT ( 'NONE',  ( -112.0284649023453198, -298.1815470323154500, -254.1601685751500668 ) ) ;
#65789=CARTESIAN_POINT ( 'NONE',  ( 39.58706461736021254, -278.0519495502701943, -270.3284710469133074 ) ) ;
#65790=CARTESIAN_POINT ( 'NONE',  ( -92.83893396777953910, -239.1568807800618686, -338.3566629249717153 ) ) ;
#65791=CARTESIAN_POINT ( 'NONE',  ( -94.37114856999372137, -286.2807001801144793, -224.2774780387568114 ) ) ;
#65792=CARTESIAN_POINT ( 'NONE',  ( -13.04916144716970194, -288.1236820990559409, -198.3621834290005097 ) ) ;
#65793=CARTESIAN_POINT ( 'NONE',  ( -39.96928640252048126, -285.3668521753272103, -197.3064230012119538 ) ) ;
#65794=CARTESIAN_POINT ( 'NONE',  ( -108.9532641653668037, -276.7185518354165765, -288.2521160139815493 ) ) ;
#65795=CARTESIAN_POINT ( 'NONE',  ( -109.5727850814231488, -286.6354750945367869, -253.1734081941833665 ) ) ;
#65796=CARTESIAN_POINT ( 'NONE',  ( -110.3055038760450799, -277.1718095932899359, -259.6640377211767259 ) ) ;
#65797=CARTESIAN_POINT ( 'NONE',  ( 24.25153651951646694, -277.1809694172739569, -310.2102383099570488 ) ) ;
#65798=CARTESIAN_POINT ( 'NONE',  ( 23.09971970921002793, -275.4738785465905266, -229.2920820922656446 ) ) ;
#65799=CARTESIAN_POINT ( 'NONE',  ( 39.30493128313072049, -286.3621550812214878, -271.5604674432495358 ) ) ;
#65800=CARTESIAN_POINT ( 'NONE',  ( 37.98926664671574116, -282.5448017530379730, -285.5072153618228867 ) ) ;
#65801=CARTESIAN_POINT ( 'NONE',  ( -50.07714253274934180, -283.7027095863974182, -346.2920567947306267 ) ) ;
#65805=CARTESIAN_POINT ( 'NONE',  ( -72.57804810807863305, -291.3739294491061855, -337.4480240295351336 ) ) ;
#65806=CARTESIAN_POINT ( 'NONE',  ( -113.5141541007331085, -289.3337913093113798, -262.6697758023958045 ) ) ;
#65808=CARTESIAN_POINT ( 'NONE',  ( -108.7517081852593464, -295.5398667591188655, -286.2737694533433910 ) ) ;
#65809=CARTESIAN_POINT ( 'NONE',  ( -42.03943701922745646, -291.3429867301673539, -193.6066780146360600 ) ) ;
#65810=CARTESIAN_POINT ( 'NONE',  ( 19.20612184350011375, -285.3674413547179256, -223.0862767112967333 ) ) ;
#65812=CARTESIAN_POINT ( 'NONE',  ( 34.38077034015644529, -288.5526976312329452, -254.7720918403955750 ) ) ;
#65813=CARTESIAN_POINT ( 'NONE',  ( -37.30987171927208124, -297.5519495502701943, -345.3611179825600175 ) ) ;
#65814=CARTESIAN_POINT ( 'NONE',  ( -40.23541020264898549, -291.0886579432597614, -345.3180200138587566 ) ) ;
#65815=CARTESIAN_POINT ( 'NONE',  ( -92.27090468178320748, -287.8345793505854431, -321.7470851548818018 ) ) ;
#65817=CARTESIAN_POINT ( 'NONE',  ( -100.6623538141222696, -292.0104403931363777, -310.6489867038565649 ) ) ;
#65818=CARTESIAN_POINT ( 'NONE',  ( -109.1620598710921115, -285.6817880712897590, -256.0347655112273060 ) ) ;
#65819=CARTESIAN_POINT ( 'NONE',  ( -93.36237009153266797, -293.2486548185485162, -220.2441252074445686 ) ) ;
#65820=CARTESIAN_POINT ( 'NONE',  ( 82.15113745099867515, -299.3754171896197818, -193.3637965294381900 ) ) ;
#65823=CARTESIAN_POINT ( 'NONE',  ( -30.66838526091325789, -300.0552191073463177, -194.7989468035448510 ) ) ;
#65825=CARTESIAN_POINT ( 'NONE',  ( 1.177652195100557853, -281.7210041291835410, -332.6204407054860894 ) ) ;
#65826=CARTESIAN_POINT ( 'NONE',  ( -81.83249319231074992, -281.6575907635549356, -330.8043033774057449 ) ) ;
#65827=CARTESIAN_POINT ( 'NONE',  ( 35.33034868849125587, -293.0663844995115710, -295.4827128101073868 ) ) ;
#65828=CARTESIAN_POINT ( 'NONE',  ( -69.91703860872395637, -271.8569159029796651, -203.9019475137396853 ) ) ;
#65829=CARTESIAN_POINT ( 'NONE',  ( 25.18081956565028889, -274.1816276034521138, -310.8572134494829697 ) ) ;
#65830=CARTESIAN_POINT ( 'NONE',  ( -75.48079136813949219, -298.8474813595877322, -207.4797142714373024 ) ) ;
#65832=CARTESIAN_POINT ( 'NONE',  ( -112.7661943181041124, -294.9089359349839583, -261.1350847545549527 ) ) ;
#65833=CARTESIAN_POINT ( 'NONE',  ( 26.31135669083326079, -295.4799752652416487, -307.2889296374409582 ) ) ;
#65835=CARTESIAN_POINT ( 'NONE',  ( -92.30524410099367572, -296.6671932431084429, -318.6478714582084422 ) ) ;
#65837=CARTESIAN_POINT ( 'NONE',  ( -111.8570138474588305, -282.7200249352006836, -258.7983972988339474 ) ) ;
#65838=CARTESIAN_POINT ( 'NONE',  ( -94.45132050873985463, -297.1942678994180937, -224.8914439131643803 ) ) ;
#65839=CARTESIAN_POINT ( 'NONE',  ( -104.4170152507197571, -284.0602523342612926, -308.2831568665051236 ) ) ;
#65840=CARTESIAN_POINT ( 'NONE',  ( 21.41915046918228072, -284.1215632595194052, -317.8839265780024448 ) ) ;
#65841=CARTESIAN_POINT ( 'NONE',  ( 14.23586249001719573, -286.4199161249086956, -213.1450519873649512 ) ) ;
#65842=CARTESIAN_POINT ( 'NONE',  ( 37.12225008550011296, -291.4499572032673882, -262.4323633119647639 ) ) ;
#65843=CARTESIAN_POINT ( 'NONE',  ( -103.2677838921256210, -278.2662545243572367, -230.7873124337938009 ) ) ;
#65844=CARTESIAN_POINT ( 'NONE',  ( 10.59707575819633618, -279.9094976428775681, -330.5268031993606428 ) ) ;
#65846=CARTESIAN_POINT ( 'NONE',  ( 4.966710597622522982, -285.4327853263189922, -210.3228458875806268 ) ) ;
#65847=CARTESIAN_POINT ( 'NONE',  ( -73.04221787564945600, -288.4343173699147087, -338.2504473885968537 ) ) ;
#65848=DIRECTION ( 'NONE',  ( -1.000000000000000000, -0.000000000000000000, -0.000000000000000000 ) ) ;
#65849=CARTESIAN_POINT ( 'NONE',  ( -88.80179633647965431, -279.1834931639543242, -326.8453174527124929 ) ) ;
#65850=CARTESIAN_POINT ( 'NONE',  ( -39.09538557066380093, -293.0941708233737018, -345.6959133537567936 ) ) ;
#65851=CARTESIAN_POINT ( 'NONE',  ( 34.50549055392714592, -281.3917765261786030, -283.4721980409929643 ) ) ;
#65852=CARTESIAN_POINT ( 'NONE',  ( 29.57572045997232735, -294.2147258880775098, -308.5615993393387271 ) ) ;
#65853=CARTESIAN_POINT ( 'NONE',  ( 2.012281269467944611, -284.6544373614743222, -205.8585727185341341 ) ) ;
#65854=CARTESIAN_POINT ( 'NONE',  ( -93.48208219091732474, -281.2440130118706065, -220.6292554365479646 ) ) ;
#65855=CARTESIAN_POINT ( 'NONE',  ( -107.6820329705125232, -295.8796896351516921, -249.9737193238597683 ) ) ;
#65858=CARTESIAN_POINT ( 'NONE',  ( 35.94439541251172443, -283.3482763720529647, -256.1166257135086539 ) ) ;
#65860=CARTESIAN_POINT ( 'NONE',  ( -85.33152481854864391, -281.1952119285918457, -330.4860931364850671 ) ) ;
#65861=CARTESIAN_POINT ( 'NONE',  ( -2.621342065655723363, -273.6966477828996744, -201.7997052641869686 ) ) ;
#65862=CARTESIAN_POINT ( 'NONE',  ( -107.7263773463444920, -290.1273863138068236, -289.9122635209611190 ) ) ;
#65863=CARTESIAN_POINT ( 'NONE',  ( -81.72070101549196863, -280.9558767872229055, -211.4649633205696944 ) ) ;
#65864=CARTESIAN_POINT ( 'NONE',  ( -90.78989565143865548, -274.8783297375145480, -219.4532258195929160 ) ) ;
#65865=CARTESIAN_POINT ( 'NONE',  ( -67.54531942401760602, -285.0419614023305712, -340.3195470548292292 ) ) ;
#65866=CARTESIAN_POINT ( 'NONE',  ( 24.45652004839766036, -280.8930520690052504, -310.0538963542088595 ) ) ;
#65867=CARTESIAN_POINT ( 'NONE',  ( -72.57172559098098930, -279.5186622458451779, -336.5862199601089060 ) ) ;
#65869=CARTESIAN_POINT ( 'NONE',  ( -15.77532429850858620, -274.1568500131879773, -196.3876383848830471 ) ) ;
#65870=CARTESIAN_POINT ( 'NONE',  ( 26.06180387523198050, -294.9438736946376025, -231.2593390296383973 ) ) ;
#65871=DIRECTION ( 'NONE',  ( 0.000000000000000000, 0.000000000000000000, -1.000000000000000000 ) ) ;
#65872=CARTESIAN_POINT ( 'NONE',  ( 14.61415361889143760, -292.4695821745240210, -325.5054263021999645 ) ) ;
#65873=CARTESIAN_POINT ( 'NONE',  ( -2.879096943440680345, -274.0283724233834732, -205.9381607116308146 ) ) ;
#65875=CARTESIAN_POINT ( 'NONE',  ( 33.80926092852174492, -294.7181304391621097, -242.6425893817074950 ) ) ;
#65876=CARTESIAN_POINT ( 'NONE',  ( 39.58706461736021254, -284.0519495502703080, -270.3284710469133074 ) ) ;
#65877=CARTESIAN_POINT ( 'NONE',  ( 8.600460027102576177, -293.8706629469612608, -208.9978884705523967 ) ) ;
#65878=CARTESIAN_POINT ( 'NONE',  ( -12.65975566729633428, -290.7306689656015237, -341.0069249568863938 ) ) ;
#65879=CARTESIAN_POINT ( 'NONE',  ( 35.00833566613925285, -273.7982598874033897, -289.4791918884091615 ) ) ;
#65880=CARTESIAN_POINT ( 'NONE',  ( -68.62066859927622886, -279.3865951612418712, -337.9246740013025487 ) ) ;
#65881=CARTESIAN_POINT ( 'NONE',  ( 19.92554231376057672, -292.2935245048903425, -317.9192628601773549 ) ) ;
#65882=CARTESIAN_POINT ( 'NONE',  ( -109.3827079970369738, -280.7144166943138544, -246.7338633729383446 ) ) ;
#65885=CARTESIAN_POINT ( 'NONE',  ( -80.64208556750783430, -283.3242018049514854, -329.2216841063703896 ) ) ;
#65886=CARTESIAN_POINT ( 'NONE',  ( -94.73960930164052741, -280.3236726324363417, -219.4988280940565915 ) ) ;
#65887=CARTESIAN_POINT ( 'NONE',  ( -31.68102171690648206, -281.7771537337149539, -346.7678083002064113 ) ) ;
#65888=CARTESIAN_POINT ( 'NONE',  ( -42.77750913042631709, -278.0604198057099552, -346.9331245745490264 ) ) ;
#65889=CARTESIAN_POINT ( 'NONE',  ( 35.91472517847984847, -276.7998691822635351, -248.8177041494605533 ) ) ;
#65890=CARTESIAN_POINT ( 'NONE',  ( -82.13390479932378696, -293.9090924074131408, -214.2458315076590907 ) ) ;
#65892=CARTESIAN_POINT ( 'NONE',  ( -63.80845765909949563, -299.7073753037106485, -200.1313016257661843 ) ) ;
#65893=CARTESIAN_POINT ( 'NONE',  ( -29.56662005178704788, -274.9734487608597533, -344.6519395095928644 ) ) ;
#65894=CARTESIAN_POINT ( 'NONE',  ( -107.4410674961157497, -292.6902660290031122, -241.0344627663689892 ) ) ;
#65895=CARTESIAN_POINT ( 'NONE',  ( 14.95422200761641562, -292.1620778603046915, -219.2099503084498622 ) ) ;
#65896=CARTESIAN_POINT ( 'NONE',  ( 18.59576727346057723, -287.7818032554592946, -323.1865535597679582 ) ) ;
#65898=CARTESIAN_POINT ( 'NONE',  ( 37.74957912682096151, -291.9486960904557122, -256.2223035354735998 ) ) ;
#65899=CARTESIAN_POINT ( 'NONE',  ( -94.92185217541755549, -282.3065766172842928, -316.5436213277922661 ) ) ;
#65900=CARTESIAN_POINT ( 'NONE',  ( -111.5397449963474230, -292.3654667848398958, -273.9926129638059251 ) ) ;
#65901=CARTESIAN_POINT ( 'NONE',  ( -92.02279969251297587, -283.7336356121102767, -220.8828702972186875 ) ) ;
#65902=CARTESIAN_POINT ( 'NONE',  ( -4.592467130376145512, -283.9264818236449059, -336.1542119788002765 ) ) ;
#65903=CARTESIAN_POINT ( 'NONE',  ( -15.00921045676239629, -289.7111584425884416, -343.8611031199193917 ) ) ;
#65904=CARTESIAN_POINT ( 'NONE',  ( -14.29540576429860188, -280.8514322604997915, -200.9761362627264702 ) ) ;
#65905=CARTESIAN_POINT ( 'NONE',  ( 19.13335302357579337, -291.6393496880280054, -218.6061463346869402 ) ) ;
#65906=CARTESIAN_POINT ( 'NONE',  ( 22.85898160912359955, -287.7144297596924503, -222.5904200343319133 ) ) ;
#65907=CARTESIAN_POINT ( 'NONE',  ( 36.63031377635126518, -287.7769118219187590, -249.0138320403187322 ) ) ;
#65908=CARTESIAN_POINT ( 'NONE',  ( -95.76721665583242782, -285.3331676562137318, -226.5951606299279888 ) ) ;
#65912=CARTESIAN_POINT ( 'NONE',  ( 37.99520844272763043, -295.3042731890324148, -261.8409060735369280 ) ) ;
#65913=CARTESIAN_POINT ( 'NONE',  ( -34.88734675084126025, -293.7067547396778195, -346.8285909597219074 ) ) ;
#65914=CARTESIAN_POINT ( 'NONE',  ( -106.4903298721224303, -277.2892350638995254, -294.6370839284992371 ) ) ;
#65916=CARTESIAN_POINT ( 'NONE',  ( -30.48752868040909192, -297.4844462213418979, -193.4637846374093613 ) ) ;
#65917=CARTESIAN_POINT ( 'NONE',  ( 25.44867885469276558, -291.5041519684930904, -231.6886148249389237 ) ) ;
#65918=CARTESIAN_POINT ( 'NONE',  ( -19.04246480916356887, -276.0509228699447135, -198.5924736606033321 ) ) ;
#65919=CARTESIAN_POINT ( 'NONE',  ( -110.7381659365240409, -294.9211031748773735, -260.4389765355931559 ) ) ;
#65920=CARTESIAN_POINT ( 'NONE',  ( 22.90513883822377039, -294.1758070528954931, -228.4170414593597798 ) ) ;
#65921=CARTESIAN_POINT ( 'NONE',  ( 28.67889141215444226, -295.0626537967168019, -302.3452616740846679 ) ) ;
#65923=CARTESIAN_POINT ( 'NONE',  ( -44.64350477871803946, -293.1440563137820732, -345.2244300709161848 ) ) ;
#65924=CARTESIAN_POINT ( 'NONE',  ( -35.76203819307012566, -300.0720829547246353, -195.3605707076006013 ) ) ;
#65925=CARTESIAN_POINT ( 'NONE',  ( -39.95440870581483495, -290.0269077196645071, -343.5995299415985187 ) ) ;
#65926=CARTESIAN_POINT ( 'NONE',  ( -72.13091536240513335, -295.8589809509435895, -334.5766211629199915 ) ) ;
#65927=CARTESIAN_POINT ( 'NONE',  ( -88.08550981830383364, -279.7380237565122911, -326.0699375581911568 ) ) ;
#65928=CARTESIAN_POINT ( 'NONE',  ( -112.8154426446185852, -277.0792615340583893, -282.8915794164530553 ) ) ;
#65929=CARTESIAN_POINT ( 'NONE',  ( 7.182734913916002384, -273.9894863080115215, -207.5989751464046549 ) ) ;
#65930=CARTESIAN_POINT ( 'NONE',  ( -21.09733145479795624, -280.9221035006244733, -343.0601076353809162 ) ) ;
#65931=CARTESIAN_POINT ( 'NONE',  ( -113.4110265899463599, -277.0083979453259531, -265.9004021971235261 ) ) ;
#65932=CARTESIAN_POINT ( 'NONE',  ( -33.97136655586751885, -278.0943049750007958, -195.2700447427622237 ) ) ;
#65934=CARTESIAN_POINT ( 'NONE',  ( -40.52266495658383860, -296.6961748250478763, -196.9242040062792967 ) ) ;
#65935=CARTESIAN_POINT ( 'NONE',  ( -41.79599345211435235, -275.9963199119455339, -195.4430843555014405 ) ) ;
#65937=CARTESIAN_POINT ( 'NONE',  ( -87.53473460053250221, -289.3757413580710818, -214.1555480570359578 ) ) ;
#65938=CARTESIAN_POINT ( 'NONE',  ( -106.5135117000522911, -290.1164061756080628, -304.3092349933458536 ) ) ;
#65939=CARTESIAN_POINT ( 'NONE',  ( -21.76028743816657141, -276.2515857240513242, -196.8271258288489776 ) ) ;
#65940=CARTESIAN_POINT ( 'NONE',  ( -108.1874836982243124, -270.8706271185409946, -245.7465776028672337 ) ) ;
#65941=CARTESIAN_POINT ( 'NONE',  ( -108.0824881141068374, -283.3651533450540114, -300.4956054416641109 ) ) ;
#65943=CARTESIAN_POINT ( 'NONE',  ( 21.18455266390713021, -280.1972415876811056, -317.2819622906920358 ) ) ;
#65945=CARTESIAN_POINT ( 'NONE',  ( -49.74078322464380619, -290.6855396640504523, -197.9673190511191763 ) ) ;
#65946=CARTESIAN_POINT ( 'NONE',  ( -24.91206906884427852, -284.3518004266574053, -197.1217259765511756 ) ) ;
#65949=CARTESIAN_POINT ( 'NONE',  ( 36.18203819356016027, -291.3618678629532610, -255.5536686649602700 ) ) ;
#65950=CARTESIAN_POINT ( 'NONE',  ( -59.41507680527886492, -278.9429034422712448, -340.7827514188816167 ) ) ;
#65951=CARTESIAN_POINT ( 'NONE',  ( -13.53071806803214194, -283.9547827405726252, -343.1693994564748209 ) ) ;
#65952=CARTESIAN_POINT ( 'NONE',  ( -3.394394904562281212, -274.6874083083788491, -337.8802947113563278 ) ) ;
#65953=CARTESIAN_POINT ( 'NONE',  ( -22.45983557658234986, -286.2478943656337833, -198.8422511808585398 ) ) ;
#65954=CARTESIAN_POINT ( 'NONE',  ( 21.31750813661597732, -277.5968364044633745, -314.7961515080252752 ) ) ;
#65955=CARTESIAN_POINT ( 'NONE',  ( -71.72104108337192940, -278.3215278409545022, -334.9559156926094374 ) ) ;
#65956=CARTESIAN_POINT ( 'NONE',  ( -75.12186625607682799, -287.5493480374124715, -205.5119532044941195 ) ) ;
#65957=VERTEX_POINT ( 'NONE', #9381 ) ;
#65959=CARTESIAN_POINT ( 'NONE',  ( -81.87343011763827860, -295.4734290814205906, -333.2428401687030259 ) ) ;
#65960=CARTESIAN_POINT ( 'NONE',  ( -51.02886567050759936, -291.2076823765269751, -343.7931668184233445 ) ) ;
#65962=CARTESIAN_POINT ( 'NONE',  ( -55.63300648810263738, -276.3376638359844719, -190.3683826091709363 ) ) ;
#65963=CARTESIAN_POINT ( 'NONE',  ( -109.3113213907166568, -277.8104039890518493, -243.7151196863976850 ) ) ;
#65964=CARTESIAN_POINT ( 'NONE',  ( 38.85679907281704715, -291.9157062107698266, -267.4873151123534853 ) ) ;
#65965=CARTESIAN_POINT ( 'NONE',  ( 24.10154053994182988, -288.5119644990451206, -229.5817167905381666 ) ) ;
#65966=CARTESIAN_POINT ( 'NONE',  ( -110.0343559269828120, -280.1303189486744714, -284.3474544559434207 ) ) ;
#65967=CARTESIAN_POINT ( 'NONE',  ( 22.83473592384047990, -289.6118616578893352, -317.4714989777941128 ) ) ;
#65968=CARTESIAN_POINT ( 'NONE',  ( -54.11278054615037547, -285.2675302830276109, -343.5154558611239963 ) ) ;
#65969=CARTESIAN_POINT ( 'NONE',  ( -114.0441001613910288, -278.8106921386081467, -263.0160367791310705 ) ) ;
#65970=CARTESIAN_POINT ( 'NONE',  ( -95.17950200455065612, -271.2084113306615905, -222.8561745852593390 ) ) ;
#65971=CARTESIAN_POINT ( 'NONE',  ( -67.36050189434993740, -279.5025040208689120, -199.4536321645202861 ) ) ;
#65972=CARTESIAN_POINT ( 'NONE',  ( -111.4231494417489756, -274.4841323063036498, -264.8448713526778420 ) ) ;
#65974=CARTESIAN_POINT ( 'NONE',  ( -106.6379572354042296, -292.6233781216987495, -303.7686719486574702 ) ) ;
#65975=CARTESIAN_POINT ( 'NONE',  ( -4.246915530093622770, -272.7222692138797697, -201.9457069542743568 ) ) ;
#65977=CARTESIAN_POINT ( 'NONE',  ( -91.33807603188630253, -278.7649825298331621, -221.1434399492984255 ) ) ;
#65978=CARTESIAN_POINT ( 'NONE',  ( 38.74506690713576518, -276.8744282527746918, -279.6842598408074423 ) ) ;
#65979=CARTESIAN_POINT ( 'NONE',  ( 95.73017409340855011, -301.1753302961462282, -196.7389390362352231 ) ) ;
#65980=CARTESIAN_POINT ( 'NONE',  ( -50.06634564565337087, -282.2693411840519957, -346.1175613297530163 ) ) ;
#65981=CARTESIAN_POINT ( 'NONE',  ( 35.28277365933605836, -289.4988292765806932, -284.6976763241843855 ) ) ;
#65982=CARTESIAN_POINT ( 'NONE',  ( -43.25551352050557341, -299.4990130816950114, -194.2312246572168135 ) ) ;
#65983=CARTESIAN_POINT ( 'NONE',  ( -103.5145756664146290, -298.2631219816349812, -231.6669218888956721 ) ) ;
#65984=CARTESIAN_POINT ( 'NONE',  ( -34.19934104096697070, -297.0126997540321554, -345.1284504759887000 ) ) ;
#65985=CARTESIAN_POINT ( 'NONE',  ( 32.79733761175518225, -279.2108490636829288, -244.1250818987050764 ) ) ;
#65986=CARTESIAN_POINT ( 'NONE',  ( -99.19224125675204107, -271.1414247475190678, -228.4795093348032822 ) ) ;
#65987=CARTESIAN_POINT ( 'NONE',  ( 33.11189621951743334, -288.7779186230117148, -241.1935299996296749 ) ) ;
#65988=CARTESIAN_POINT ( 'NONE',  ( 1.463601776810747435, -287.4404803334741700, -332.5573768527789298 ) ) ;
#65989=CARTESIAN_POINT ( 'NONE',  ( 123.0373869404028113, 148.7393932779486079, -263.4038933679887577 ) ) ;
#65991=CARTESIAN_POINT ( 'NONE',  ( -2.088830972431062971, -287.1693679847561498, -338.1537540920544984 ) ) ;
#65992=CARTESIAN_POINT ( 'NONE',  ( -66.34133048055761606, -289.1091883054617142, -337.4308879379889277 ) ) ;
#65994=CARTESIAN_POINT ( 'NONE',  ( -70.94324956237295510, -286.6988010066888251, -201.4232591024590135 ) ) ;
#65995=CARTESIAN_POINT ( 'NONE',  ( -16.37073773745650129, -277.1069362282830753, -340.3591661227330292 ) ) ;
#65996=CARTESIAN_POINT ( 'NONE',  ( 8.676474224327343165, -291.5862835011914740, -208.9448498506494616 ) ) ;
#65997=CARTESIAN_POINT ( 'NONE',  ( -16.16193853528575630, -283.4368465355158264, -344.3401479676193730 ) ) ;
#65998=CARTESIAN_POINT ( 'NONE',  ( 30.46993938637740484, -283.5273767765294792, -305.3509636138021506 ) ) ;
#65999=CARTESIAN_POINT ( 'NONE',  ( 2.086954024954835507, -282.8726163968291303, -336.4756059801734978 ) ) ;
#66000=CARTESIAN_POINT ( 'NONE',  ( 20.53008303935344969, -281.2586714350285320, -225.8105357819634662 ) ) ;
#66001=CARTESIAN_POINT ( 'NONE',  ( 65.15629269179825656, 47.80519856837923243, -319.0222192987535550 ) ) ;
#66002=CARTESIAN_POINT ( 'NONE',  ( -54.34637575705281876, -279.2711085221470739, -343.2902765430991963 ) ) ;
#66003=CARTESIAN_POINT ( 'NONE',  ( 166.9140850792291531, 232.6971882099037146, -192.2382519929172418 ) ) ;
#66004=CARTESIAN_POINT ( 'NONE',  ( -77.96030328704325996, -207.4903925274613243, -353.7115950856197628 ) ) ;
#66005=CARTESIAN_POINT ( 'NONE',  ( -102.1687970221487234, -272.2111267290140404, -236.3390446985912661 ) ) ;
#66006=CARTESIAN_POINT ( 'NONE',  ( 37.70267676728949624, -292.8467791220786580, -253.3353416622107090 ) ) ;
#66007=CARTESIAN_POINT ( 'NONE',  ( 168.1374001855827771, 229.6528827650084850, -190.0556063141613663 ) ) ;
#66008=CARTESIAN_POINT ( 'NONE',  ( 6.963136212523474811, -273.3258323534875558, -207.9231837627890229 ) ) ;
#66009=CARTESIAN_POINT ( 'NONE',  ( -20.97148885136189733, -287.2384240427127793, -342.3226118230091970 ) ) ;
#66010=CARTESIAN_POINT ( 'NONE',  ( -10.01361473381519929, -296.5519072661414839, -339.3831523595944759 ) ) ;
#66011=CARTESIAN_POINT ( 'NONE',  ( 33.86221415781191979, -288.6281075565840410, -252.1102026907373670 ) ) ;
#66012=ORIENTED_EDGE ( 'NONE', *, *, #72819, .F. ) ;
#66013=CARTESIAN_POINT ( 'NONE',  ( -19.33081930196000187, -295.7672974475588035, -345.0377406702301073 ) ) ;
#66014=CARTESIAN_POINT ( 'NONE',  ( -41.33255420213366449, -286.4929353506379357, -197.3961484234209820 ) ) ;
#66015=CARTESIAN_POINT ( 'NONE',  ( -34.10243567483509963, -273.0123313599640937, -193.7386690775432498 ) ) ;
#66016=CARTESIAN_POINT ( 'NONE',  ( -27.75781637311466810, -295.7363576475738682, -346.6527932587918599 ) ) ;
#66017=CARTESIAN_POINT ( 'NONE',  ( 32.12770106494478739, -293.6188855934028084, -237.1687736219842293 ) ) ;
#66018=CARTESIAN_POINT ( 'NONE',  ( -107.3958945317856148, -290.9909506204559193, -249.7884584224612183 ) ) ;
#66020=CARTESIAN_POINT ( 'NONE',  ( -55.02086467013484850, -275.7466931561976935, -196.8984653198138801 ) ) ;
#66021=CARTESIAN_POINT ( 'NONE',  ( -0.2243317157130767237, -273.3294074106844960, -203.3364276961902135 ) ) ;
#66024=CARTESIAN_POINT ( 'NONE',  ( -99.37453220276103139, -278.6649973889156513, -224.8256493548919082 ) ) ;
#66025=CARTESIAN_POINT ( 'NONE',  ( -33.75048651690141099, -296.5777826597361013, -196.6687291552181591 ) ) ;
#66026=CARTESIAN_POINT ( 'NONE',  ( -68.57837650279431330, -275.6066369441006145, -337.7185155995596233 ) ) ;
#66027=CARTESIAN_POINT ( 'NONE',  ( -38.09929201648341035, -275.1221121905756490, -197.0559194685275202 ) ) ;
#66028=CARTESIAN_POINT ( 'NONE',  ( -62.12054311311919008, -274.6631157985659115, -201.4451010611083746 ) ) ;
#66029=CARTESIAN_POINT ( 'NONE',  ( -73.48292372479861001, -275.3399509485612953, -203.4611192335009093 ) ) ;
#66030=CARTESIAN_POINT ( 'NONE',  ( 32.20547296823256289, -273.1937361781164668, -241.2159385632868407 ) ) ;
#66031=CARTESIAN_POINT ( 'NONE',  ( -106.0802043782211115, -296.8708493983693870, -295.3878298224027503 ) ) ;
#66032=CARTESIAN_POINT ( 'NONE',  ( 28.91724979246798455, -292.5581131290470580, -302.4961697213598200 ) ) ;
#66034=CARTESIAN_POINT ( 'NONE',  ( -45.63674563646462445, -277.6468202138307788, -346.9041275316455426 ) ) ;
#66035=CARTESIAN_POINT ( 'NONE',  ( -11.49220680197487354, -274.5650069652637626, -202.0369934768249323 ) ) ;
#66036=CARTESIAN_POINT ( 'NONE',  ( -111.4018388592818098, -282.9946217862026856, -289.6066973615876350 ) ) ;
#66037=CARTESIAN_POINT ( 'NONE',  ( -109.4492848898728852, -298.2790390378648908, -291.6320294789139211 ) ) ;
#66039=CARTESIAN_POINT ( 'NONE',  ( 2.543587831087332329, -285.7992832856398877, -209.0278844860571894 ) ) ;
#66041=CARTESIAN_POINT ( 'NONE',  ( -111.1678542005621324, -276.8604487981932039, -265.1006059854234422 ) ) ;
#66042=CARTESIAN_POINT ( 'NONE',  ( -108.3938765661287817, -276.8758715650670297, -289.5174000258427327 ) ) ;
#66043=CARTESIAN_POINT ( 'NONE',  ( -8.246032400199567292, -284.6713510151253104, -339.5011695459937755 ) ) ;
#66044=CARTESIAN_POINT ( 'NONE',  ( 3.136201015468592868, -275.8139566337198971, -209.0740009697422863 ) ) ;
#66046=CARTESIAN_POINT ( 'NONE',  ( 38.75671217578710070, -273.8907332383798803, -265.5112157061028597 ) ) ;
#66047=CARTESIAN_POINT ( 'NONE',  ( -81.19052702700666657, -281.4579206195212464, -209.3094283791246539 ) ) ;
#66049=CARTESIAN_POINT ( 'NONE',  ( 13.26396962234478494, -288.6729886025011638, -214.1805127963725113 ) ) ;
#66050=CARTESIAN_POINT ( 'NONE',  ( 37.69313454270169217, -291.5317616071852171, -268.7859035075917404 ) ) ;
#66052=CARTESIAN_POINT ( 'NONE',  ( -110.0682975175384257, -271.3802467245080265, -259.4268275758536788 ) ) ;
#66053=CARTESIAN_POINT ( 'NONE',  ( -41.64108055106496664, -290.1371457672456131, -196.1998288687785532 ) ) ;
#66054=CARTESIAN_POINT ( 'NONE',  ( 192.1331913634949160, 286.0196433216794389, -110.9393339982713940 ) ) ;
#66055=CARTESIAN_POINT ( 'NONE',  ( -40.57949923632136802, -296.0112990352631073, -195.4181424580750104 ) ) ;
#66056=CARTESIAN_POINT ( 'NONE',  ( 25.79468216994817098, -285.4616420928705907, -227.4833052941875735 ) ) ;
#66057=CARTESIAN_POINT ( 'NONE',  ( 21.66165175352695371, -283.7681958806242619, -314.7108346939210151 ) ) ;
#66058=CARTESIAN_POINT ( 'NONE',  ( -30.94650066090903096, -284.3717522162310729, -194.6309231019361903 ) ) ;
#66059=CARTESIAN_POINT ( 'NONE',  ( -74.07530136059953918, -284.9753751873201963, -334.1845109833982974 ) ) ;
#66061=CARTESIAN_POINT ( 'NONE',  ( -53.71588573135835532, -284.0703950441616712, -341.7189099582902827 ) ) ;
#66062=CARTESIAN_POINT ( 'NONE',  ( -38.86117933839373251, -291.0510151458734640, -345.7010011079727292 ) ) ;
#66063=CARTESIAN_POINT ( 'NONE',  ( -90.15144164196092902, -273.6634804787148596, -214.2805050641428863 ) ) ;
#66065=CARTESIAN_POINT ( 'NONE',  ( 2.401529393632486187, -286.6042686961881145, -334.6859261543385742 ) ) ;
#66066=CARTESIAN_POINT ( 'NONE',  ( 27.64882962133886579, -276.0944812524138570, -311.7546724988639539 ) ) ;
#66067=CARTESIAN_POINT ( 'NONE',  ( 32.35536109802747262, -295.1829867537711038, -243.6372249810924586 ) ) ;
#66069=CARTESIAN_POINT ( 'NONE',  ( -95.95921662488163406, -292.4090924074130839, -317.1477375740089997 ) ) ;
#66070=CARTESIAN_POINT ( 'NONE',  ( -34.84646163410921815, -281.7050120358837262, -343.8244200158424633 ) ) ;
#66071=CARTESIAN_POINT ( 'NONE',  ( -76.87292535886210487, -275.5796475827423251, -334.3536929904196313 ) ) ;
#66072=CARTESIAN_POINT ( 'NONE',  ( -111.7627580636821705, -271.2447935318899681, -253.5024735639898097 ) ) ;
#66073=CARTESIAN_POINT ( 'NONE',  ( 11.81011439785202022, -275.6966483520877205, -324.5407205639933181 ) ) ;
#66074=CARTESIAN_POINT ( 'NONE',  ( 13.36634690950409521, -294.2975295354068521, -216.8877440760342665 ) ) ;
#66075=CARTESIAN_POINT ( 'NONE',  ( -2.337482997635717652, -293.4686188073713424, -206.0187097626381956 ) ) ;
#66076=CARTESIAN_POINT ( 'NONE',  ( -109.3566275938010364, -286.5352166089218713, -253.2235999723304474 ) ) ;
#66077=CARTESIAN_POINT ( 'NONE',  ( 34.93503741262060203, -295.2941302456838457, -295.3161050383188808 ) ) ;
#66078=CARTESIAN_POINT ( 'NONE',  ( 21.91537591650899586, -295.5212637591776570, -318.7748427327967988 ) ) ;
#66079=CARTESIAN_POINT ( 'NONE',  ( -110.0994113897043150, -296.2992449649553919, -276.8975311389967260 ) ) ;
#66080=CARTESIAN_POINT ( 'NONE',  ( -70.84354940306981518, -291.4942087385542777, -337.4769689093386660 ) ) ;
#66081=CARTESIAN_POINT ( 'NONE',  ( -34.47684589114251708, -283.1837523824060554, -347.3078048165201608 ) ) ;
#66082=CARTESIAN_POINT ( 'NONE',  ( -34.79486249015194232, -296.1636494873990273, -194.8019355729566371 ) ) ;
#66083=CARTESIAN_POINT ( 'NONE',  ( -49.34263412137227789, -285.7366782149577489, -194.2483421608772574 ) ) ;
#66084=CARTESIAN_POINT ( 'NONE',  ( -73.61982333243398102, -279.5159652989553365, -335.6118894819285288 ) ) ;
#66085=CARTESIAN_POINT ( 'NONE',  ( -41.32924030689272854, -284.7957865902727690, -197.0598755493348619 ) ) ;
#66086=CARTESIAN_POINT ( 'NONE',  ( 31.03089293745648192, -285.9562495446321577, -301.1862564772725364 ) ) ;
#66087=CARTESIAN_POINT ( 'NONE',  ( -88.08631184020785554, -277.4904669211045984, -214.1002091699997436 ) ) ;
#66089=CARTESIAN_POINT ( 'NONE',  ( -89.70258657129043911, -284.7967025947124853, -219.3343681353435670 ) ) ;
#66090=CARTESIAN_POINT ( 'NONE',  ( 3.596731780877818530, -281.7944765932532505, -205.5523993004658792 ) ) ;
#66091=CARTESIAN_POINT ( 'NONE',  ( -20.55955531734109698, -287.9006213800693672, -345.3234250713186952 ) ) ;
#66093=CARTESIAN_POINT ( 'NONE',  ( -5.599255531615181525, -278.2417037915337801, -339.6349054416850777 ) ) ;
#66094=CARTESIAN_POINT ( 'NONE',  ( -45.57976181540851712, -278.4695144073904771, -346.4758676100841512 ) ) ;
#66095=CARTESIAN_POINT ( 'NONE',  ( -96.40445346122366743, -278.9858919640156500, -227.4590064584303661 ) ) ;
#66096=CARTESIAN_POINT ( 'NONE',  ( -92.35136436181264230, -275.2403398427313164, -219.8864300158642493 ) ) ;
#66097=CARTESIAN_POINT ( 'NONE',  ( 8.850926610725585064, -292.6657811484924423, -208.6890426982433269 ) ) ;
#66098=CARTESIAN_POINT ( 'NONE',  ( 32.00407513567640905, -285.9353487869912556, -298.1230440207729089 ) ) ;
#66099=CARTESIAN_POINT ( 'NONE',  ( -8.829665107975266380, -294.0191345196998896, -199.6963865043881583 ) ) ;
#66100=CARTESIAN_POINT ( 'NONE',  ( -26.17382344825159279, -293.8269501812651470, -342.8145830715150169 ) ) ;
#66101=CARTESIAN_POINT ( 'NONE',  ( -38.34684057618156316, -294.7318136091298015, -343.3753438536031126 ) ) ;
#66102=CARTESIAN_POINT ( 'NONE',  ( -101.4332290556287717, -292.1887592232049542, -228.1496667420828999 ) ) ;
#66103=CARTESIAN_POINT ( 'NONE',  ( 35.62109070840234892, -282.1441816992916642, -265.8529230820548150 ) ) ;
#66105=CARTESIAN_POINT ( 'NONE',  ( -92.99330366548598192, -272.3359316672772366, -217.4673774189938058 ) ) ;
#66106=CARTESIAN_POINT ( 'NONE',  ( 37.40729431877169731, -288.4302970889677908, -288.4694880668265569 ) ) ;
#66107=CARTESIAN_POINT ( 'NONE',  ( 20.64905750427460518, -280.3590095926362551, -319.1194763697392887 ) ) ;
#66108=CARTESIAN_POINT ( 'NONE',  ( 35.92892959339673808, -288.1823469417914225, -293.9653360743826624 ) ) ;
#66109=CARTESIAN_POINT ( 'NONE',  ( -2.179929660692826676, -286.8641446966494755, -206.3064384258233019 ) ) ;
#66111=CARTESIAN_POINT ( 'NONE',  ( 23.82377260802752517, -22.69053332001751855, -342.9562588441870048 ) ) ;
#66112=CARTESIAN_POINT ( 'NONE',  ( 121.1859076339088261, 147.6349627520604315, -260.2004405834634326 ) ) ;
#66113=CARTESIAN_POINT ( 'NONE',  ( -106.4200512936071448, -277.4276321675980626, -294.6142659312679370 ) ) ;
#66114=CARTESIAN_POINT ( 'NONE',  ( -89.31462926828430682, -276.7250682024576918, -322.1346745910945515 ) ) ;
#66115=CARTESIAN_POINT ( 'NONE',  ( 19.33869485627723961, -298.2516321568845115, -193.4272256200833056 ) ) ;
#66116=CARTESIAN_POINT ( 'NONE',  ( 66.48133663197175736, 45.91875831897123561, -316.4011423777610617 ) ) ;
#66117=CARTESIAN_POINT ( 'NONE',  ( 24.08057763346275593, -295.9141664115978756, -315.1186874849448145 ) ) ;
#66118=CARTESIAN_POINT ( 'NONE',  ( -33.51147481886336266, -292.5939780942691186, -197.3875446723942844 ) ) ;
#66119=CARTESIAN_POINT ( 'NONE',  ( -96.76159264080231992, -274.1480947809783970, -221.7391969496065656 ) ) ;
#66120=CARTESIAN_POINT ( 'NONE',  ( 8.273016916975223012, -287.0975865961645468, -327.9852541188967052 ) ) ;
#66121=CARTESIAN_POINT ( 'NONE',  ( -85.75050163867139474, -274.0532577059026380, -210.6124717838628158 ) ) ;
#66122=CARTESIAN_POINT ( 'NONE',  ( -71.66687781941519120, -297.7519742814442907, -205.9203557116978232 ) ) ;
#66125=CARTESIAN_POINT ( 'NONE',  ( -111.8212895134480647, -280.6345699979332267, -257.6290731998062711 ) ) ;
#66126=CARTESIAN_POINT ( 'NONE',  ( -89.29522423156527111, -278.8840629922526091, -322.1541459818229214 ) ) ;
#66127=CARTESIAN_POINT ( 'NONE',  ( -105.4273245950790141, -279.8715159360588700, -304.2184560779058415 ) ) ;
#66128=CARTESIAN_POINT ( 'NONE',  ( -1.367413542175457408, -273.0182866451992822, -206.0305844135806126 ) ) ;
#66131=CARTESIAN_POINT ( 'NONE',  ( -74.50761706514632010, -279.7099112787716422, -207.4723333888128138 ) ) ;
#66132=CARTESIAN_POINT ( 'NONE',  ( 38.97844609957957118, -276.4722499455084517, -279.7180645430580626 ) ) ;
#66133=CARTESIAN_POINT ( 'NONE',  ( 34.96443898096862313, -277.8090652615731528, -290.3294791407587354 ) ) ;
#66134=CARTESIAN_POINT ( 'NONE',  ( -103.1079713876986688, -276.6150240926625088, -309.3674106093390037 ) ) ;
#66137=CARTESIAN_POINT ( 'NONE',  ( 37.04826314654771835, -283.6867148496959885, -282.4643720260480677 ) ) ;
#66138=CARTESIAN_POINT ( 'NONE',  ( -9.656915403891026983, -291.6203586457856431, -202.5860582337112419 ) ) ;
#66139=CARTESIAN_POINT ( 'NONE',  ( -37.97327468512063575, -285.3930244844734148, -193.4656441189118823 ) ) ;
#66140=CARTESIAN_POINT ( 'NONE',  ( -56.60392223614617535, -281.5437258422837203, -341.8239811392599563 ) ) ;
#66141=CARTESIAN_POINT ( 'NONE',  ( 10.27626711274774784, -280.9551496881786079, -326.5343017521307161 ) ) ;
#66142=CARTESIAN_POINT ( 'NONE',  ( 34.45038752060246878, -282.5561904310054615, -255.0360839601250689 ) ) ;
#66144=CARTESIAN_POINT ( 'NONE',  ( -34.52911555161163903, -281.4172295406225430, -346.5091959951091667 ) ) ;
#66145=CARTESIAN_POINT ( 'NONE',  ( -111.9509851454597111, -298.4541466758237220, -278.0067204115215418 ) ) ;
#66146=CARTESIAN_POINT ( 'NONE',  ( -29.67585023549577983, -288.1491791819337891, -195.5863684260210675 ) ) ;
#66148=CARTESIAN_POINT ( 'NONE',  ( -67.77170110816078363, -293.5760985054318439, -201.1854005458759787 ) ) ;
#66149=CARTESIAN_POINT ( 'NONE',  ( 19.81654992031413087, -274.2240834862521979, -318.9196919231536071 ) ) ;
#66151=CARTESIAN_POINT ( 'NONE',  ( -51.66524851583518796, -288.4280885383340660, -345.8528048202717855 ) ) ;
#66152=CARTESIAN_POINT ( 'NONE',  ( 29.47135571708405521, -291.5317990336986327, -238.8962851691227911 ) ) ;
#66153=CARTESIAN_POINT ( 'NONE',  ( -109.6140389296505617, -277.4117689209807622, -257.0212333084846250 ) ) ;
#66154=CARTESIAN_POINT ( 'NONE',  ( -93.13440738901661575, -294.0043750418785748, -319.3308974227988415 ) ) ;
#66155=CARTESIAN_POINT ( 'NONE',  ( -95.32940307620039277, -291.2351964166499556, -315.5330746465203333 ) ) ;
#66158=CARTESIAN_POINT ( 'NONE',  ( 3.836708363788984499, -292.9888542598583285, -334.6654121107679885 ) ) ;
#66159=CARTESIAN_POINT ( 'NONE',  ( -1.819014711898614634, -288.1307872994415220, -205.6154633439350619 ) ) ;
#66160=CARTESIAN_POINT ( 'NONE',  ( -93.94134525835545446, -289.4889604077101239, -219.6614711810919687 ) ) ;
#66161=CARTESIAN_POINT ( 'NONE',  ( -76.16431008742902975, -291.0074205110040566, -332.8765550575475345 ) ) ;
#66164=CARTESIAN_POINT ( 'NONE',  ( -29.14490234459867324, -289.7484541362188111, -343.0619723992427907 ) ) ;
#66166=CARTESIAN_POINT ( 'NONE',  ( 27.11901448957914340, -289.3040594959810505, -311.8452425603758797 ) ) ;
#66167=CARTESIAN_POINT ( 'NONE',  ( -76.61333355973137316, -277.5499408138261970, -205.9878486124086692 ) ) ;
#66168=CARTESIAN_POINT ( 'NONE',  ( -84.55731244321239615, -279.7555171181150513, -209.4953843830671474 ) ) ;
#66169=CARTESIAN_POINT ( 'NONE',  ( -22.56607903649278413, -279.9029110658683521, -194.7593732424615780 ) ) ;
#66170=CARTESIAN_POINT ( 'NONE',  ( -9.997698658045548470, -284.4089916776244991, -200.5095058365575085 ) ) ;
#66171=CARTESIAN_POINT ( 'NONE',  ( 82.64890176555634582, -299.5541904835127980, -195.3611179825600175 ) ) ;
#66172=CARTESIAN_POINT ( 'NONE',  ( -16.55349886411488924, -278.4632098133459408, -199.0960061382260449 ) ) ;
#66173=CARTESIAN_POINT ( 'NONE',  ( -3.810469677352952722, -280.6097109925814834, -337.4623265507131578 ) ) ;
#66175=CARTESIAN_POINT ( 'NONE',  ( -106.9516383514800992, -276.6277249140856611, -301.7493912487947227 ) ) ;
#66176=CARTESIAN_POINT ( 'NONE',  ( -109.9365306865469591, -283.1596655254510893, -295.0893020166682277 ) ) ;
#66177=CARTESIAN_POINT ( 'NONE',  ( -37.16102936435173376, -298.9957304702170973, -197.1229343357308323 ) ) ;
#66178=CARTESIAN_POINT ( 'NONE',  ( -76.14923425061607531, -274.9698771563925561, -204.4776238346569244 ) ) ;
#66179=CARTESIAN_POINT ( 'NONE',  ( 0.8788775508262285374, -276.1940202473241470, -332.6400997886959772 ) ) ;
#66180=CARTESIAN_POINT ( 'NONE',  ( -98.01168189571093592, -297.9514028555648224, -314.4755901044721895 ) ) ;
#66181=CARTESIAN_POINT ( 'NONE',  ( -78.13460596832146621, -289.7508380882433698, -335.7298134849900748 ) ) ;
#66182=CARTESIAN_POINT ( 'NONE',  ( -22.81854561775204360, -278.3162935493934356, -196.1567302363904446 ) ) ;
#66183=CARTESIAN_POINT ( 'NONE',  ( -77.16744560436603706, -291.3675513776994990, -204.3988677873917652 ) ) ;
#66184=CARTESIAN_POINT ( 'NONE',  ( -71.29245107400900849, -288.5706700674882654, -335.2656172880286363 ) ) ;
#66185=CARTESIAN_POINT ( 'NONE',  ( 37.60729084355889995, -291.5874995104225036, -273.1268725211789956 ) ) ;
#66188=CARTESIAN_POINT ( 'NONE',  ( -110.0334865253988283, -290.1565627107095793, -263.0199578598904964 ) ) ;
#66190=CARTESIAN_POINT ( 'NONE',  ( -12.79034058128880602, -287.3049248243992793, -197.6283814949794930 ) ) ;
#66191=CARTESIAN_POINT ( 'NONE',  ( -21.33282851196159058, -297.3376638359844719, -340.3538533559490702 ) ) ;
#66192=ADVANCED_FACE ( 'NONE', ( #26409 ), #40118, .F. ) ;
#66193=CARTESIAN_POINT ( 'NONE',  ( 23.83418438494624070, -293.2306099254367382, -316.7327835532024096 ) ) ;
#66194=CARTESIAN_POINT ( 'NONE',  ( 13.36654357170882967, -283.6755981805604847, -327.7201503939587042 ) ) ;
#66195=CARTESIAN_POINT ( 'NONE',  ( -94.12070177419889205, -285.0345505328479021, -224.4594481924937099 ) ) ;
#66196=CARTESIAN_POINT ( 'NONE',  ( 27.06065995135497104, -276.3856676272631034, -234.8491716076192688 ) ) ;
#66197=CARTESIAN_POINT ( 'NONE',  ( 28.59953159782821785, -292.0395868346770385, -305.4515059461646160 ) ) ;
#66198=CARTESIAN_POINT ( 'NONE',  ( -72.08219691047548849, -272.3772148180811428, -205.6498068435246580 ) ) ;
#66200=CARTESIAN_POINT ( 'NONE',  ( -113.2098679957031493, -271.2709011634024137, -296.4525692007673570 ) ) ;
#66201=CARTESIAN_POINT ( 'NONE',  ( -22.10588334872066341, -294.5288140447204341, -345.8171593477336501 ) ) ;
#66202=CARTESIAN_POINT ( 'NONE',  ( 17.00947126192458114, -288.7544643511031950, -219.4771558312718582 ) ) ;
#66203=CARTESIAN_POINT ( 'NONE',  ( -110.5223253264944532, -297.9231711942348966, -247.2483553638753619 ) ) ;
#66204=CARTESIAN_POINT ( 'NONE',  ( -19.79941697596794370, -286.9351261977479908, -199.3952038431443725 ) ) ;
#66205=CARTESIAN_POINT ( 'NONE',  ( -103.2035382961771717, -278.1278574104970858, -230.8238118596773063 ) ) ;
#66206=CARTESIAN_POINT ( 'NONE',  ( -24.91609755745417232, -295.5491945781254799, -346.3026428160024466 ) ) ;
#66207=CARTESIAN_POINT ( 'NONE',  ( 20.52996379649732361, -286.3613126322387075, -319.2607703108955661 ) ) ;
#66208=CARTESIAN_POINT ( 'NONE',  ( 19.51693187456766410, -294.5918196319122444, -322.3313484280354260 ) ) ;
#66209=CARTESIAN_POINT ( 'NONE',  ( -2.433060018909899203, -292.8607462158156522, -206.2105460648086250 ) ) ;
#66211=FACE_BOUND ( 'NONE', #56522, .T. ) ;
#66212=CARTESIAN_POINT ( 'NONE',  ( 197.0305496340489526, 281.6334632708399681, -110.2979370532489725 ) ) ;
#66213=CARTESIAN_POINT ( 'NONE',  ( 38.65864648130963133, -289.1584726103948242, -277.1915694142041389 ) ) ;
#66214=CARTESIAN_POINT ( 'NONE',  ( 40.65961533371913106, -290.8380690714489560, -252.5904736702033802 ) ) ;
#66217=CARTESIAN_POINT ( 'NONE',  ( -56.52319810575206560, -279.1599330881629157, -195.8388643604391746 ) ) ;
#66218=CARTESIAN_POINT ( 'NONE',  ( 33.08850524321100295, -283.8826458234749452, -295.8050803148556156 ) ) ;
#66219=CARTESIAN_POINT ( 'NONE',  ( -61.45241253695066064, -183.8721261770043611, -361.2693405134621685 ) ) ;
#66221=CARTESIAN_POINT ( 'NONE',  ( -95.35719787236388356, -283.8037644705867137, -220.5544399037451342 ) ) ;
#66222=CARTESIAN_POINT ( 'NONE',  ( -20.83331738389067667, -286.9184498722517560, -342.9475319595702558 ) ) ;
#66223=CARTESIAN_POINT ( 'NONE',  ( -5.652821940133198275, -276.3248819761196842, -201.5416404841618032 ) ) ;
#66224=CARTESIAN_POINT ( 'NONE',  ( -57.92811876987593678, -298.2712828428845455, -200.2598497414804228 ) ) ;
#66225=CARTESIAN_POINT ( 'NONE',  ( -58.56655815169438029, -294.0172417464543173, -340.7226762288333930 ) ) ;
#66226=CARTESIAN_POINT ( 'NONE',  ( -112.8975821993737867, -279.3835805932195058, -255.9860603205730172 ) ) ;
#66227=CARTESIAN_POINT ( 'NONE',  ( 33.89326580096770414, -275.7633822261303749, -286.3735107259606139 ) ) ;
#66228=CARTESIAN_POINT ( 'NONE',  ( 25.88191826893634584, -276.0563511635842247, -226.9297079082920732 ) ) ;
#66229=CARTESIAN_POINT ( 'NONE',  ( -1.623932807737227701, -275.5102978981704496, -338.2266733710313815 ) ) ;
#66231=CARTESIAN_POINT ( 'NONE',  ( 37.17849715955711076, -273.4376097656809748, -261.4529637872618082 ) ) ;
#66232=CARTESIAN_POINT ( 'NONE',  ( -112.0253742975123572, -297.7738308010550554, -286.5152229647271156 ) ) ;
#66235=CARTESIAN_POINT ( 'NONE',  ( -71.33370899889742134, -286.6718353107985422, -205.4090633014450304 ) ) ;
#66236=CARTESIAN_POINT ( 'NONE',  ( -80.96128524120030079, -285.3952042039550179, -332.6449365984241808 ) ) ;
#66237=CARTESIAN_POINT ( 'NONE',  ( -2.130011946789559296, -285.8796093435105377, -206.2416184379708000 ) ) ;
#66238=CARTESIAN_POINT ( 'NONE',  ( -109.3832904801213033, -277.1616709541115711, -254.2892951371272261 ) ) ;
#66239=CARTESIAN_POINT ( 'NONE',  ( -104.1134967517435967, -285.9792942613892137, -302.9196978354106022 ) ) ;
#66240=CARTESIAN_POINT ( 'NONE',  ( -111.0439562123325032, -277.0646320494101360, -267.8656547143996249 ) ) ;
#66241=CARTESIAN_POINT ( 'NONE',  ( -24.26099852445735650, -277.9610216637191229, -342.5454526789682177 ) ) ;
#66243=CARTESIAN_POINT ( 'NONE',  ( -110.4032385894416564, -273.0444201342810402, -270.3673720632041864 ) ) ;
#66244=CARTESIAN_POINT ( 'NONE',  ( 37.51785605277983393, -282.1371794258329260, -252.9768987208467763 ) ) ;
#66245=CARTESIAN_POINT ( 'NONE',  ( -4.184672242022903887, -283.1190158340443759, -339.8028128101969969 ) ) ;
#66249=CARTESIAN_POINT ( 'NONE',  ( 26.09046235596253283, -288.8593408859181295, -228.9284467850930582 ) ) ;
#66250=CARTESIAN_POINT ( 'NONE',  ( -111.0712337495254616, -288.9794200432615412, -290.7879176716971870 ) ) ;
#66251=CARTESIAN_POINT ( 'NONE',  ( -109.0450232749765433, -295.5571919200965567, -284.9574814036002408 ) ) ;
#66252=CARTESIAN_POINT ( 'NONE',  ( -73.37859312159817193, -290.9355723273632748, -202.4149856994655750 ) ) ;
#66253=CARTESIAN_POINT ( 'NONE',  ( -15.66602171189749804, -287.2465526226158090, -340.8479028432313385 ) ) ;
#66254=CARTESIAN_POINT ( 'NONE',  ( 23.99063488775317410, -286.6869393951224083, -311.0500775808962999 ) ) ;
#66256=CARTESIAN_POINT ( 'NONE',  ( -38.64727948680960168, -287.2405332112700762, -196.9631070599960196 ) ) ;
#66257=CARTESIAN_POINT ( 'NONE',  ( -108.6402299844791628, -276.8544628302163346, -246.9258729306777411 ) ) ;
#66258=CARTESIAN_POINT ( 'NONE',  ( -34.71078962606990359, -291.0192456420278404, -345.3149635237269308 ) ) ;
#66259=CARTESIAN_POINT ( 'NONE',  ( -59.51144153415526006, -287.3384259627416100, -342.1840320860181350 ) ) ;
#66260=CARTESIAN_POINT ( 'NONE',  ( -95.29530733418177135, -284.8647811227368152, -315.1564422041469129 ) ) ;
#66261=CARTESIAN_POINT ( 'NONE',  ( -110.5379609001591916, -292.7713613690945067, -253.2632865322329110 ) ) ;
#66264=CARTESIAN_POINT ( 'NONE',  ( -107.6414661936025396, -274.8849138503065319, -243.0815948640712065 ) ) ;
#66265=CARTESIAN_POINT ( 'NONE',  ( 27.93006829711379879, -280.3002559186471103, -237.2003369834671105 ) ) ;
#66266=CARTESIAN_POINT ( 'NONE',  ( 17.26502906607845489, -280.2731301445279541, -321.8471598800334732 ) ) ;
#66267=CARTESIAN_POINT ( 'NONE',  ( 29.42927706732763582, -293.2453693709277900, -308.4921940707182557 ) ) ;
#66268=CARTESIAN_POINT ( 'NONE',  ( -90.91483488503378396, -271.5186021575332234, -219.2750459673879391 ) ) ;
#66269=CARTESIAN_POINT ( 'NONE',  ( -29.58726449603378938, -275.0331772571075248, -344.4480384772639354 ) ) ;
#66270=CARTESIAN_POINT ( 'NONE',  ( -55.43113996832510537, -299.1298088578427041, -199.0763255000922527 ) ) ;
#66272=CARTESIAN_POINT ( 'NONE',  ( -113.3244589239191953, -294.8017813316301954, -269.5901594478612537 ) ) ;
#66274=CARTESIAN_POINT ( 'NONE',  ( -28.80978810612744567, -296.3672858384592246, -343.5055084722031893 ) ) ;
#66276=CARTESIAN_POINT ( 'NONE',  ( -68.57701191593261569, -296.2762252371691716, -336.5334537720560775 ) ) ;
#66279=CARTESIAN_POINT ( 'NONE',  ( -99.62253987202920769, -283.1449827732726021, -227.8484269787984999 ) ) ;
#66280=CARTESIAN_POINT ( 'NONE',  ( -103.7185893734331330, -296.9633585651827161, -239.8567469666458578 ) ) ;
#66281=CARTESIAN_POINT ( 'NONE',  ( -110.9260302234101516, -284.8390000856119855, -247.5024510225785548 ) ) ;
#66282=CARTESIAN_POINT ( 'NONE',  ( 37.01301151980471360, -283.6445369452757177, -283.8752483961154667 ) ) ;
#66283=CARTESIAN_POINT ( 'NONE',  ( -49.33724514145076512, -285.5701039007482223, -194.2689122834692625 ) ) ;
#66284=CARTESIAN_POINT ( 'NONE',  ( 36.72586583802087290, -291.4145776740485871, -259.6829112690270449 ) ) ;
#66285=CARTESIAN_POINT ( 'NONE',  ( -112.6954123733869579, -277.7079001701363836, -285.7602027750559159 ) ) ;
#66286=CARTESIAN_POINT ( 'NONE',  ( -106.6662871844225293, -281.6237833571633473, -303.7098442033569654 ) ) ;
#66288=CARTESIAN_POINT ( 'NONE',  ( 31.76814765271049978, -286.6744077386492791, -295.0787117998168014 ) ) ;
#66290=CARTESIAN_POINT ( 'NONE',  ( -84.98345390722781190, -288.6120137024563519, -330.5267680774360315 ) ) ;
#66291=FACE_OUTER_BOUND ( 'NONE', #71598, .T. ) ;
#66292=CARTESIAN_POINT ( 'NONE',  ( -112.4206482094779176, -280.1573145912028053, -256.0869066622111632 ) ) ;
#66293=CARTESIAN_POINT ( 'NONE',  ( 3.318125674472236497, -292.5291581139214259, -333.8668899640919108 ) ) ;
#66294=CARTESIAN_POINT ( 'NONE',  ( 21.02424669222132536, -281.8350989828747970, -314.2623411900966062 ) ) ;
#66295=CARTESIAN_POINT ( 'NONE',  ( 0.5423524140913242864, -294.7283853601740589, -337.4120983849635991 ) ) ;
#66296=CARTESIAN_POINT ( 'NONE',  ( -29.58597057095891714, -284.2294967350505317, -195.2002048942119643 ) ) ;
#66297=CARTESIAN_POINT ( 'NONE',  ( -104.3991098286895323, -280.9972328294093700, -236.6551308134961005 ) ) ;
#66298=CARTESIAN_POINT ( 'NONE',  ( -110.6495100021942335, -270.7648327654998184, -253.7480675990668715 ) ) ;
#66301=CARTESIAN_POINT ( 'NONE',  ( 36.66007489787520512, -283.4009729962876349, -260.2010829297898908 ) ) ;
#66302=CARTESIAN_POINT ( 'NONE',  ( -77.98917990656750021, -295.1221123911157065, -331.1327783948392494 ) ) ;
#66303=CARTESIAN_POINT ( 'NONE',  ( 121.3395553409046670, -299.5541904835127980, -195.3611179825600175 ) ) ;
#66304=CARTESIAN_POINT ( 'NONE',  ( -112.3417001280813707, -270.0523547857347353, -270.3292895737510548 ) ) ;
#66305=CARTESIAN_POINT ( 'NONE',  ( -64.83274058808314066, -272.8992798406845282, -198.5946004532373763 ) ) ;
#66307=CARTESIAN_POINT ( 'NONE',  ( -98.84290870578105626, -289.8415005164987406, -309.6879707422454544 ) ) ;
#66308=CARTESIAN_POINT ( 'NONE',  ( -79.46690301104561627, -280.9916952213127956, -209.8948047739962419 ) ) ;
#66309=CARTESIAN_POINT ( 'NONE',  ( -11.22598392839584136, -275.9982241095415247, -201.2817819423349590 ) ) ;
#66310=CARTESIAN_POINT ( 'NONE',  ( -21.86832297695727689, -284.4571705894740603, -344.9735500094316762 ) ) ;
#66311=CARTESIAN_POINT ( 'NONE',  ( -54.57119190547125243, -278.6208465729222326, -198.9624758551673551 ) ) ;
#66312=CARTESIAN_POINT ( 'NONE',  ( -65.04893841182567371, -279.4141527832276779, -340.1106632695494909 ) ) ;
#66314=CARTESIAN_POINT ( 'NONE',  ( -81.24864485088895094, -273.3070385659617614, -207.0416248235253533 ) ) ;
#66315=CARTESIAN_POINT ( 'NONE',  ( -97.94772280539935139, -293.0654984960622187, -227.0509325671463614 ) ) ;
#66316=DIRECTION ( 'NONE',  ( 0.000000000000000000, 0.000000000000000000, -1.000000000000000000 ) ) ;
#66317=CARTESIAN_POINT ( 'NONE',  ( 38.37164501064047784, -291.7272215707329224, -273.1530430956136684 ) ) ;
#66319=CARTESIAN_POINT ( 'NONE',  ( 21.53448887771002163, -274.4541891647140801, -227.0993240997837574 ) ) ;
#66320=CARTESIAN_POINT ( 'NONE',  ( -37.81037309103371058, -293.5664969595428602, -194.0558881400799294 ) ) ;
#66321=CARTESIAN_POINT ( 'NONE',  ( 35.78497577281001440, -278.2662352645559167, -287.0191576251351080 ) ) ;
#66322=CARTESIAN_POINT ( 'NONE',  ( 19.11260001187631730, -294.0491121035935862, -218.5835097482835181 ) ) ;
#66324=CARTESIAN_POINT ( 'NONE',  ( 3.424946345996064068, -288.6018247239894094, -207.6067638692849471 ) ) ;
#66325=CARTESIAN_POINT ( 'NONE',  ( 18.79403842591196749, -274.2415484329758328, -319.8658665008601929 ) ) ;
#66326=B_SPLINE_CURVE_WITH_KNOTS ( 'NONE', 3,
 ( #9267, #23021, #46190, #75095, #1259, #51900, #23504, #31995, #39073, #15941, #44795, #38144, #8807, #67061, #60427, #2197, #89267, #24417, #53297, #82647, #32476, #10675, #68929, #62290 ),
 .UNSPECIFIED., .F., .F.,
 ( 4, 2, 2, 2, 2, 2, 2, 2, 2, 2, 2, 4 ),
 ( 5.000000000000000311E-10, 0.06250000043739496747, 0.1250000003747899491, 0.2500000002495798568, 0.3750000001243697922, 0.4999999999991597277, 0.6249999998739497187, 0.7499999997487397652, 0.8124999996861348439, 0.8749999996235298116, 0.9374999995609247794, 0.9999999994983197471 ),
 .UNSPECIFIED. ) ;
#66327=CARTESIAN_POINT ( 'NONE',  ( 36.04115808835049251, -277.3096142734244154, -257.7847379865123116 ) ) ;
#66328=CARTESIAN_POINT ( 'NONE',  ( 37.14883234711485471, -291.6375679589755237, -270.7921943464806986 ) ) ;
#66329=CARTESIAN_POINT ( 'NONE',  ( -98.44595379486447939, -281.0173802862722710, -225.5443959811486820 ) ) ;
#66331=CARTESIAN_POINT ( 'NONE',  ( -33.49935557264054609, -282.6692078668725685, -343.2936768864429951 ) ) ;
#66332=CARTESIAN_POINT ( 'NONE',  ( -50.89854609281908893, -280.9624848078023547, -194.8779779019191380 ) ) ;
#66333=CARTESIAN_POINT ( 'NONE',  ( -81.34607319154994798, -282.4304646125908675, -333.1283203970305067 ) ) ;
#66334=CARTESIAN_POINT ( 'NONE',  ( -41.36010559900251593, -278.0428033818589029, -347.0337453539904686 ) ) ;
#66335=CARTESIAN_POINT ( 'NONE',  ( 24.75134548844062010, -276.4791412284788521, -225.9860788277405845 ) ) ;
#66336=CARTESIAN_POINT ( 'NONE',  ( 30.89617123739170168, -283.8376638359844719, -254.7536222014695397 ) ) ;
#66337=ORIENTED_EDGE ( 'NONE', *, *, #14901, .T. ) ;
#66338=CARTESIAN_POINT ( 'NONE',  ( -108.9583337159623966, -274.8347243186335618, -248.4788891605057870 ) ) ;
#66339=CARTESIAN_POINT ( 'NONE',  ( -14.76420760042905655, -293.4313878049808864, -200.6152729145111095 ) ) ;
#66340=CARTESIAN_POINT ( 'NONE',  ( -111.7975396809801651, -276.6407332248783746, -265.0531280738588293 ) ) ;
#66341=CARTESIAN_POINT ( 'NONE',  ( -37.47698575588407266, -290.8139219892755705, -346.3605677252420492 ) ) ;
#66342=CARTESIAN_POINT ( 'NONE',  ( 4.568863140731014738, -291.9827902628720722, -210.4041752620166790 ) ) ;
#66343=CARTESIAN_POINT ( 'NONE',  ( 22.35342337738662621, -287.7117428803312009, -318.9206914852170485 ) ) ;
#66345=CARTESIAN_POINT ( 'NONE',  ( -110.4013569069839491, -283.0880799951265203, -259.9338955989343276 ) ) ;
#66346=CARTESIAN_POINT ( 'NONE',  ( -111.3521065996476835, -292.3295727306268645, -276.7595594117125870 ) ) ;
#66347=CARTESIAN_POINT ( 'NONE',  ( -101.5863601767124607, -283.5226122734850378, -234.1549068759208012 ) ) ;
#66348=CARTESIAN_POINT ( 'NONE',  ( -35.66824909721538717, -281.3887259151706530, -196.8745333958138417 ) ) ;
#66349=CARTESIAN_POINT ( 'NONE',  ( -99.67218712236601164, -290.8974015767936976, -315.1913412864594193 ) ) ;
#66350=CARTESIAN_POINT ( 'NONE',  ( -57.13590006197910043, -280.2821311035039002, -200.0320479583949975 ) ) ;
#66351=CARTESIAN_POINT ( 'NONE',  ( -37.77729363036129229, -290.8417404348701325, -193.7594275390628127 ) ) ;
#66352=CARTESIAN_POINT ( 'NONE',  ( 31.27300087953015151, -287.9089917782112025, -235.7752592302306880 ) ) ;
#66353=CARTESIAN_POINT ( 'NONE',  ( -3.082497158390807179, -289.1041096724353565, -339.2657485101670432 ) ) ;
#66354=CARTESIAN_POINT ( 'NONE',  ( -59.98064433010927132, -285.9171105684835652, -200.9602663313739299 ) ) ;
#66357=CARTESIAN_POINT ( 'NONE',  ( 36.55127138825917399, -295.1991612316996907, -253.5658206663924261 ) ) ;
#66358=CARTESIAN_POINT ( 'NONE',  ( -25.00395213005931794, -293.5829239540091748, -345.9203204897705746 ) ) ;
#66359=CARTESIAN_POINT ( 'NONE',  ( -1.365063887643188645, -275.6216248807390343, -334.2079192884575036 ) ) ;
#66360=CARTESIAN_POINT ( 'NONE',  ( -43.27360506565078424, -297.3278282692725156, -193.6390453134878555 ) ) ;
#66361=CARTESIAN_POINT ( 'NONE',  ( 15.38498961005499943, -291.2935091543484987, -218.8039926352263933 ) ) ;
#66362=CARTESIAN_POINT ( 'NONE',  ( -108.5842135590440591, -294.5304442075395173, -290.4229796823129277 ) ) ;
#66363=CARTESIAN_POINT ( 'NONE',  ( -1.073747979820776077, -293.7500094523796861, -206.5361733068681644 ) ) ;
#66364=CARTESIAN_POINT ( 'NONE',  ( 34.51677014748355532, -294.4412016062966018, -255.8495252330793619 ) ) ;
#66366=CARTESIAN_POINT ( 'NONE',  ( -33.55333369635184226, -293.0044396248879934, -345.4450694999377447 ) ) ;
#66367=CARTESIAN_POINT ( 'NONE',  ( 27.29300515917568148, -300.8614267717341022, -195.3390746317473088 ) ) ;
#66368=CARTESIAN_POINT ( 'NONE',  ( -109.1671486716764861, -291.3045187041875579, -284.7260276395792289 ) ) ;
#66369=CARTESIAN_POINT ( 'NONE',  ( -80.16374633245293069, -295.9834818402999304, -329.5080523541774937 ) ) ;
#66370=CARTESIAN_POINT ( 'NONE',  ( -94.67122848778222988, -281.2062132988971825, -221.4359537063214134 ) ) ;
#66371=CARTESIAN_POINT ( 'NONE',  ( -53.63899006283128301, -278.5322222808999300, -195.5560037588437581 ) ) ;
#66373=CARTESIAN_POINT ( 'NONE',  ( -110.9371423211469931, -272.1830232205388711, -247.8851359201196658 ) ) ;
#66374=CARTESIAN_POINT ( 'NONE',  ( 34.33961225689883179, -279.8922357795186144, -290.4385594123805276 ) ) ;
#66375=CARTESIAN_POINT ( 'NONE',  ( -70.86410080892369479, -278.0171472278371425, -201.9309413702808342 ) ) ;
#66376=CARTESIAN_POINT ( 'NONE',  ( -103.1753293625201024, -277.0333375185752516, -234.0849317754581875 ) ) ;
#66377=CARTESIAN_POINT ( 'NONE',  ( 52.44288484880080148, -297.8839743961142403, -196.8885969919342642 ) ) ;
#66381=CARTESIAN_POINT ( 'NONE',  ( -110.6681626797553548, -288.3496113813343982, -287.7840965609291288 ) ) ;
#66382=CARTESIAN_POINT ( 'NONE',  ( -112.5653432347661465, -290.3464978709251341, -286.8050687778560359 ) ) ;
#66383=CARTESIAN_POINT ( 'NONE',  ( -43.90859531930468052, -275.9696206022821912, -195.4298133591807130 ) ) ;
#66384=CARTESIAN_POINT ( 'NONE',  ( -84.42694655853519237, -271.4038055238236780, -211.9832093679705451 ) ) ;
#66385=CARTESIAN_POINT ( 'NONE',  ( -95.21985270194804230, -283.0643773297090888, -320.9009861604972116 ) ) ;
#66387=CARTESIAN_POINT ( 'NONE',  ( -44.82435747161934358, -281.1465808093095120, -345.0378756386635359 ) ) ;
#66389=CARTESIAN_POINT ( 'NONE',  ( 36.01868852669803545, -292.3166263472769515, -268.0407990168725973 ) ) ;
#66390=CARTESIAN_POINT ( 'NONE',  ( -49.60259615746537776, -284.0338749568397247, -197.0930699730296283 ) ) ;
#66393=CARTESIAN_POINT ( 'NONE',  ( -19.57432356220730441, -290.2803447609423984, -197.4423248559728279 ) ) ;
#66394=CARTESIAN_POINT ( 'NONE',  ( -48.71119869762767252, -278.7993323017034868, -343.3320294535976700 ) ) ;
#66395=CARTESIAN_POINT ( 'NONE',  ( -27.40830629665333618, -284.1338210319679547, -346.3703525756164936 ) ) ;
#66396=CARTESIAN_POINT ( 'NONE',  ( -32.74530106327306100, -272.1894717146834068, -194.9281410629301661 ) ) ;
#66397=CARTESIAN_POINT ( 'NONE',  ( -54.75633926039605370, -285.8221506931667477, -199.4164344587780988 ) ) ;
#66398=CARTESIAN_POINT ( 'NONE',  ( 18.76937238010619424, -277.6489623735701571, -317.9733271361920401 ) ) ;
#66399=CARTESIAN_POINT ( 'NONE',  ( -41.85635686782941889, -277.9132939323004052, -343.3957910124282762 ) ) ;
#66400=CARTESIAN_POINT ( 'NONE',  ( -107.4247345445486843, -286.2035275346000844, -297.2146699692959260 ) ) ;
#66401=ORIENTED_EDGE ( 'NONE', *, *, #87430, .T. ) ;
#66403=CARTESIAN_POINT ( 'NONE',  ( -66.92640102486173248, -295.2626021873625177, -341.4650200683968819 ) ) ;
#66404=CARTESIAN_POINT ( 'NONE',  ( -22.14916247711017760, -288.2274679733395146, -197.2256968131548263 ) ) ;
#66406=CARTESIAN_POINT ( 'NONE',  ( 40.65961533371913106, -290.8380690714489560, -252.5904736702033802 ) ) ;
#66407=CARTESIAN_POINT ( 'NONE',  ( -113.4086810581186882, -277.6001355830888428, -260.1951521424682028 ) ) ;
#66408=CARTESIAN_POINT ( 'NONE',  ( -98.54969839028463241, -289.5620170710945445, -224.9518089885522443 ) ) ;
#66409=CARTESIAN_POINT ( 'NONE',  ( -109.0959934856486058, -285.8521682315225689, -287.2099122023921041 ) ) ;
#66410=CARTESIAN_POINT ( 'NONE',  ( -100.3419038568832207, -280.8417284533395559, -231.4181145263924861 ) ) ;
#66411=CARTESIAN_POINT ( 'NONE',  ( 39.11318161578627439, -288.9920798421018162, -271.5240665824787811 ) ) ;
#66412=CARTESIAN_POINT ( 'NONE',  ( 36.53280121039472306, -283.3861069353757784, -257.4166712002287909 ) ) ;
#66413=CARTESIAN_POINT ( 'NONE',  ( 12.70622787710087565, -276.5429018825201979, -328.8778242028647583 ) ) ;
#66414=CARTESIAN_POINT ( 'NONE',  ( -99.81056001969753311, -295.1271678595230128, -229.4082545889327491 ) ) ;
#66415=CARTESIAN_POINT ( 'NONE',  ( -93.07228700772414243, -279.1125913604073503, -217.1520707403757342 ) ) ;
#66416=CARTESIAN_POINT ( 'NONE',  ( -36.48664548758041803, -299.9830890439129121, -195.9208274694676390 ) ) ;
#66419=CARTESIAN_POINT ( 'NONE',  ( -37.30987171927208124, -279.5519495502701943, -345.3611179825600175 ) ) ;
#66420=CARTESIAN_POINT ( 'NONE',  ( -46.73324378088730668, -272.1743328474673262, -194.9570536345238736 ) ) ;
#66422=CARTESIAN_POINT ( 'NONE',  ( -109.6818351608113176, -278.1994185451076191, -259.7685426337143895 ) ) ;
#66423=CARTESIAN_POINT ( 'NONE',  ( 12.45817665826460363, -277.5811304314962058, -328.5674835242627978 ) ) ;
#66424=CARTESIAN_POINT ( 'NONE',  ( -101.2299964412172528, -283.0479968938050774, -313.0136063724921200 ) ) ;
#66425=CARTESIAN_POINT ( 'NONE',  ( 21.99918749449010491, -289.9246533858199655, -314.6161867917600716 ) ) ;
#66426=CARTESIAN_POINT ( 'NONE',  ( -35.51225111912538779, -299.5947782959736401, -194.0539833116449699 ) ) ;
#66427=CARTESIAN_POINT ( 'NONE',  ( -35.49928932413877192, -299.2798060552077573, -193.7578199242622645 ) ) ;
#66428=CARTESIAN_POINT ( 'NONE',  ( 33.52927831415468773, -295.2389984394819749, -246.1722224118713314 ) ) ;
#66429=CARTESIAN_POINT ( 'NONE',  ( 25.66050301481099893, -280.0980954985886342, -310.8388866879950569 ) ) ;
#66430=CARTESIAN_POINT ( 'NONE',  ( -10.88415542613376985, -272.4187809568127818, -200.5072420580083588 ) ) ;
#66431=CARTESIAN_POINT ( 'NONE',  ( -87.24160528045565854, -286.9707023451973100, -212.7027079817666504 ) ) ;
#66432=CARTESIAN_POINT ( 'NONE',  ( 16.22748109302714070, -287.1899460208875894, -320.4810471324510104 ) ) ;
#66433=CARTESIAN_POINT ( 'NONE',  ( 155.3377760462712445, 206.0000123873846292, -217.0427545417765032 ) ) ;
#66435=CARTESIAN_POINT ( 'NONE',  ( 36.92737983449001149, -286.3539476226549709, -288.3804692032369985 ) ) ;
#66436=CARTESIAN_POINT ( 'NONE',  ( 1.319180486372797612, -288.1867502374390142, -332.3080613846667575 ) ) ;
#66438=CARTESIAN_POINT ( 'NONE',  ( -49.31010628200724000, -286.9828289858222092, -194.5563607979073026 ) ) ;
#66439=CARTESIAN_POINT ( 'NONE',  ( 33.91483296102150291, -276.0966094320498883, -286.3739913341262309 ) ) ;
#66441=CARTESIAN_POINT ( 'NONE',  ( 35.18956090077695364, -292.7895902999543978, -295.4377947591495399 ) ) ;
#66442=CARTESIAN_POINT ( 'NONE',  ( 4.497204700011000256, -283.1553272494535918, -334.9439668628541540 ) ) ;
#66443=CARTESIAN_POINT ( 'NONE',  ( 30.09988783270704715, -282.6058122709053464, -234.5506230181639182 ) ) ;
#66444=CARTESIAN_POINT ( 'NONE',  ( 19.77067678675773266, -282.5871612583490560, -322.0522926998226012 ) ) ;
#66446=CARTESIAN_POINT ( 'NONE',  ( -14.30623014153881201, -280.6923918672146101, -201.0151350796725751 ) ) ;
#66447=CARTESIAN_POINT ( 'NONE',  ( -105.5795714935544112, -294.2666405000204009, -254.7536222014695397 ) ) ;
#66448=CARTESIAN_POINT ( 'NONE',  ( 194.6022636468435110, 278.9903764957075509, -125.9409043586979209 ) ) ;
#66450=CARTESIAN_POINT ( 'NONE',  ( -110.5532232720421462, -280.3529109491770441, -285.8563207669483859 ) ) ;
#66451=CARTESIAN_POINT ( 'NONE',  ( -13.87141369607328301, -91.16939480456166223, -359.4227886527972942 ) ) ;
#66452=CARTESIAN_POINT ( 'NONE',  ( -111.2570529628670215, -268.0638518741617986, -295.3521300423831235 ) ) ;
#66453=CARTESIAN_POINT ( 'NONE',  ( -110.4862351550085151, -295.8863065711019544, -271.4563773625523595 ) ) ;
#66454=CARTESIAN_POINT ( 'NONE',  ( 33.27040466433985699, -292.6701675038814301, -239.8085802835533684 ) ) ;
#66455=CARTESIAN_POINT ( 'NONE',  ( -110.5520430423103448, -271.6439828081399241, -270.3495548111940820 ) ) ;
#66456=CARTESIAN_POINT ( 'NONE',  ( 7.576521399050904826, -297.1788500536419519, -193.9609729414230230 ) ) ;
#66457=CARTESIAN_POINT ( 'NONE',  ( -97.21950132061779470, -288.3552761995064770, -313.5014626807680997 ) ) ;
#66458=CARTESIAN_POINT ( 'NONE',  ( -83.10291939514574722, -297.5462449141708703, -328.8798386925689101 ) ) ;
#66459=CARTESIAN_POINT ( 'NONE',  ( 19.88873418501042067, -288.2195641263478478, -224.2334746198176560 ) ) ;
#66461=CARTESIAN_POINT ( 'NONE',  ( -0.8075652796476866513, -295.5203950504831028, -337.8894923163524595 ) ) ;
#66462=CARTESIAN_POINT ( 'NONE',  ( -79.34978597921673327, -285.9605087977898847, -210.5218419567632679 ) ) ;
#66463=CARTESIAN_POINT ( 'NONE',  ( -35.46848148622010655, -296.8700448510948036, -193.7585612416910976 ) ) ;
#66464=CARTESIAN_POINT ( 'NONE',  ( -90.68121765459423500, -292.1222409655414936, -214.9785416743855251 ) ) ;
#66465=CARTESIAN_POINT ( 'NONE',  ( 37.69989018066195285, -293.8313140517606712, -253.3230648666520040 ) ) ;
#66467=CARTESIAN_POINT ( 'NONE',  ( -109.7004112790123713, -290.8511441086107538, -260.3312183724216311 ) ) ;
#66470=CARTESIAN_POINT ( 'NONE',  ( 0.4535464150409347361, -276.4717381111614714, -204.9180421043208469 ) ) ;
#66471=CARTESIAN_POINT ( 'NONE',  ( 37.56039170075763423, -274.1445016512689676, -254.2464691009641058 ) ) ;
#66473=CARTESIAN_POINT ( 'NONE',  ( 3.463544080642186440, -276.0271454067687955, -335.6500424881484150 ) ) ;
#66474=CARTESIAN_POINT ( 'NONE',  ( -38.07003196200111717, -272.4427462068400700, -196.5647091927194481 ) ) ;
#66475=CARTESIAN_POINT ( 'NONE',  ( -60.13504490293512106, -281.6141142164237294, -199.6575674739028727 ) ) ;
#66476=CARTESIAN_POINT ( 'NONE',  ( -18.72975919936687816, -274.9495012294592016, -342.2253033075599546 ) ) ;
#66477=CARTESIAN_POINT ( 'NONE',  ( -98.10708992559519004, -274.2004947042232175, -229.2608562051539138 ) ) ;
#66478=CARTESIAN_POINT ( 'NONE',  ( -48.92443079987220500, -274.8423769140602531, -197.9962336114622019 ) ) ;
#66479=CARTESIAN_POINT ( 'NONE',  ( -65.86787885169044898, -275.4442033553438591, -199.9182238212333402 ) ) ;
#66480=CARTESIAN_POINT ( 'NONE',  ( -86.93452339649391547, -271.3865157570705264, -213.5558957347547562 ) ) ;
#66481=CARTESIAN_POINT ( 'NONE',  ( -94.84849385212076811, -296.5680316617691687, -315.4927182660333642 ) ) ;
#66482=CARTESIAN_POINT ( 'NONE',  ( 35.79038758835083911, -292.2398906598892836, -278.9975681299496841 ) ) ;
#66485=CARTESIAN_POINT ( 'NONE',  ( 22.59701001507071538, -276.6916989883891347, -318.6196825054826718 ) ) ;
#66486=CARTESIAN_POINT ( 'NONE',  ( 15.44532235868296866, -274.9907889820449896, -219.8644380348377183 ) ) ;
#66487=CARTESIAN_POINT ( 'NONE',  ( -100.5793658247346229, -283.8095936837894442, -227.2060260905129496 ) ) ;
#66488=CARTESIAN_POINT ( 'NONE',  ( -107.7119898544983982, -298.2082499067275876, -296.9284819815736682 ) ) ;
#66490=CARTESIAN_POINT ( 'NONE',  ( 0.2604114106753362967, -285.7636028412070459, -207.5431242034451031 ) ) ;
#66491=CARTESIAN_POINT ( 'NONE',  ( -96.40707171369399475, -277.4102245005706209, -225.7390138244824698 ) ) ;
#66492=CARTESIAN_POINT ( 'NONE',  ( -67.05710276042545104, -276.0242310646790997, -337.6839949623957864 ) ) ;
#66493=CARTESIAN_POINT ( 'NONE',  ( 34.58704563722467640, -283.8264306477723267, -291.6487622513163842 ) ) ;
#66494=CARTESIAN_POINT ( 'NONE',  ( 34.28411631165699447, -276.9682628140044471, -286.4455762975343873 ) ) ;
#66496=CARTESIAN_POINT ( 'NONE',  ( 33.98021069235073099, -273.6090891243063083, -243.5352824689463205 ) ) ;
#66497=CARTESIAN_POINT ( 'NONE',  ( -39.55931662244956470, -282.0245547066186305, -195.2144272685848989 ) ) ;
#66499=CARTESIAN_POINT ( 'NONE',  ( -84.63107619886696398, -287.3265379459054429, -211.4287066457472406 ) ) ;
#66500=CARTESIAN_POINT ( 'NONE',  ( -94.98446313033487343, -287.8892222012290745, -318.3632743255333253 ) ) ;
#66501=CARTESIAN_POINT ( 'NONE',  ( 82.12401493620129145, -301.5056145204703171, -195.8476787650543258 ) ) ;
#66502=CARTESIAN_POINT ( 'NONE',  ( -52.70329859634396286, -296.6459803833660658, -198.5374274384009539 ) ) ;
#66503=CARTESIAN_POINT ( 'NONE',  ( -64.50183602250376680, -289.8334230107046210, -201.2590630098414124 ) ) ;
#66504=CARTESIAN_POINT ( 'NONE',  ( -79.37448608631180491, -205.8233151019928755, -350.8497528714748341 ) ) ;
#66506=CARTESIAN_POINT ( 'NONE',  ( 26.85095983609733139, -286.5793011421721985, -311.7139331892660152 ) ) ;
#66507=CARTESIAN_POINT ( 'NONE',  ( -106.9882521355795149, -283.1860748371248633, -239.8432679973196571 ) ) ;
#66508=CARTESIAN_POINT ( 'NONE',  ( -57.65494131097599961, -291.7825971754450052, -200.1913941367027974 ) ) ;
#66509=CARTESIAN_POINT ( 'NONE',  ( 13.73108449473622450, -282.2099691721807062, -217.3095081051319255 ) ) ;
#66510=CARTESIAN_POINT ( 'NONE',  ( 3.488797392179261880, -283.2906668567015345, -331.1304941987315829 ) ) ;
#66511=CARTESIAN_POINT ( 'NONE',  ( -62.19682020397199551, -291.3535493450925173, -341.5543945126098038 ) ) ;
#66513=CARTESIAN_POINT ( 'NONE',  ( -37.25571840298405135, -298.2198816790711362, -193.3603518727142898 ) ) ;
#66515=CARTESIAN_POINT ( 'NONE',  ( -70.03850431079013106, -287.5592570848596097, -338.4945918141465881 ) ) ;
#66516=CARTESIAN_POINT ( 'NONE',  ( 29.09594759657340290, -276.0587965248112141, -309.2846194285332331 ) ) ;
#66518=CARTESIAN_POINT ( 'NONE',  ( 3.111170379154164056, -294.5778371256207606, -207.5670376179971299 ) ) ;
#66520=CARTESIAN_POINT ( 'NONE',  ( 21.31550574532285580, -284.6948066931273615, -317.0979686699210447 ) ) ;
#66521=CARTESIAN_POINT ( 'NONE',  ( -79.22626523709432433, -275.6153139136299615, -332.8394249949083701 ) ) ;
#66523=CARTESIAN_POINT ( 'NONE',  ( -111.5316412369251680, -294.7315912071073853, -287.8041955825242439 ) ) ;
#66524=CARTESIAN_POINT ( 'NONE',  ( 30.36931392717984934, -275.2708971366317883, -298.0477452263011742 ) ) ;
#66525=CARTESIAN_POINT ( 'NONE',  ( -97.90780328148092337, -291.4925754448390194, -312.3648817795429409 ) ) ;
#66526=CARTESIAN_POINT ( 'NONE',  ( -99.91885982448586390, -292.0156976170268308, -232.3149942361840772 ) ) ;
#66527=CARTESIAN_POINT ( 'NONE',  ( -103.9144633109148543, -285.8790356856410995, -302.8213076755470752 ) ) ;
#66528=CARTESIAN_POINT ( 'NONE',  ( 33.90677886897459103, -294.6232960429947525, -242.6059220584592708 ) ) ;
#66529=CARTESIAN_POINT ( 'NONE',  ( 39.21811721119787819, -294.8664747357288434, -270.2935693556833030 ) ) ;
#66530=CARTESIAN_POINT ( 'NONE',  ( 12.35332046792512450, -294.1704580053282712, -323.9038025302235155 ) ) ;
#66531=CARTESIAN_POINT ( 'NONE',  ( 19.35369671610927611, -290.2339909428848159, -319.5371026280207616 ) ) ;
#66532=CARTESIAN_POINT ( 'NONE',  ( -50.09141791109876607, -283.3770948579393121, -346.3521030884660945 ) ) ;
#66533=CARTESIAN_POINT ( 'NONE',  ( -104.5028619447186173, -271.1527953924508552, -235.1809469547474691 ) ) ;
#66534=CARTESIAN_POINT ( 'NONE',  ( -99.78972236026685039, -283.7871752351571217, -315.4973625877774452 ) ) ;
#66536=CARTESIAN_POINT ( 'NONE',  ( -110.7164244104488802, -283.3040410710634092, -273.6406560215482386 ) ) ;
#66537=CARTESIAN_POINT ( 'NONE',  ( 29.88316102465614321, -285.9920934734542470, -303.7320165516460975 ) ) ;
#66538=CARTESIAN_POINT ( 'NONE',  ( -94.95092859298588905, -277.3665260073635750, -221.1326401466070024 ) ) ;
#66539=CARTESIAN_POINT ( 'NONE',  ( 197.0349383350915105, 285.8449894349855640, -111.9383547020201064 ) ) ;
#66540=CARTESIAN_POINT ( 'NONE',  ( -59.99175983336060369, -285.2581894993325591, -200.8991626623587479 ) ) ;
#66541=CARTESIAN_POINT ( 'NONE',  ( -69.27040478109327637, -288.5207737621898900, -340.1850828346537128 ) ) ;
#66542=CARTESIAN_POINT ( 'NONE',  ( -14.80663321872071414, -278.3651990363064783, -343.2079281468933800 ) ) ;
#66543=CARTESIAN_POINT ( 'NONE',  ( -20.22006829968976405, -278.1519357152525913, -344.9818892261909582 ) ) ;
#66544=CARTESIAN_POINT ( 'NONE',  ( -93.08882614292124913, -279.0554556474177730, -223.2116671916093651 ) ) ;
#66545=CARTESIAN_POINT ( 'NONE',  ( -59.99835590321384871, -275.7371306236574355, -199.1837045198811040 ) ) ;
#66546=CARTESIAN_POINT ( 'NONE',  ( 17.33086569621237771, -284.8347823811419630, -219.2448528056791019 ) ) ;
#66547=CARTESIAN_POINT ( 'NONE',  ( -106.9917741021248077, -291.7522190346152229, -301.3988668028130178 ) ) ;
#66548=CARTESIAN_POINT ( 'NONE',  ( -42.42482450855411713, -294.0380902419025233, -343.4937913948334085 ) ) ;
#66550=CARTESIAN_POINT ( 'NONE',  ( -31.60492727441741678, -294.6445953116143528, -343.2066915103906126 ) ) ;
#66551=CARTESIAN_POINT ( 'NONE',  ( -64.29310352260451111, -292.7883705282490041, -198.5060406575162517 ) ) ;
#66552=CARTESIAN_POINT ( 'NONE',  ( 18.90923190084793504, -281.5421454768553531, -223.6541646988366381 ) ) ;
#66554=CARTESIAN_POINT ( 'NONE',  ( -34.04958490837677942, -297.0127962974689808, -193.6708147898868333 ) ) ;
#66555=CARTESIAN_POINT ( 'NONE',  ( 5.116474773709787094, -287.2610284032228378, -206.1836121535922075 ) ) ;
#66556=CARTESIAN_POINT ( 'NONE',  ( -75.64947500029836647, -289.8821706816476649, -337.1313110021119996 ) ) ;
#66557=CARTESIAN_POINT ( 'NONE',  ( -10.74622434378185787, -286.7420567776412668, -202.3419405886913580 ) ) ;
#66559=CARTESIAN_POINT ( 'NONE',  ( -113.9111842188364676, -271.2735285581878202, -270.3448380411595622 ) ) ;
#66560=CARTESIAN_POINT ( 'NONE',  ( 196.2181823052468701, 281.8870305299420806, -110.2198146774690173 ) ) ;
#66561=CARTESIAN_POINT ( 'NONE',  ( -61.85353664513819183, -276.5760912380897025, -339.3480755774759245 ) ) ;
#66562=CARTESIAN_POINT ( 'NONE',  ( -70.60529391094118523, -276.4219086716603897, -335.6892084426448264 ) ) ;
#66563=CARTESIAN_POINT ( 'NONE',  ( -90.14526775557085614, -272.9970254716726572, -214.2746923727137300 ) ) ;
#66564=CARTESIAN_POINT ( 'NONE',  ( -87.51707661104852320, -230.5351160159351878, -345.2162280226144162 ) ) ;
#66565=CARTESIAN_POINT ( 'NONE',  ( -107.1331604661673111, -276.8326398854349577, -301.8341558931759323 ) ) ;
#66566=CARTESIAN_POINT ( 'NONE',  ( 33.51477028915017797, -295.6646396652234330, -297.8080597423184486 ) ) ;
#66567=CARTESIAN_POINT ( 'NONE',  ( -94.34285458221397391, -291.6900755765959161, -224.6372224042051471 ) ) ;
#66568=CARTESIAN_POINT ( 'NONE',  ( -110.6621322215138576, -297.6463770327770249, -247.2004727337939869 ) ) ;
#66569=CARTESIAN_POINT ( 'NONE',  ( -85.01758769131480165, -288.4107559172310857, -326.3590920367963122 ) ) ;
#66570=CARTESIAN_POINT ( 'NONE',  ( -93.10397136821094932, -273.9283399552204514, -217.3902058459342754 ) ) ;
#66571=CARTESIAN_POINT ( 'NONE',  ( -79.72977094586097735, -297.6276265469426789, -210.9283706387506925 ) ) ;
#66574=CARTESIAN_POINT ( 'NONE',  ( -112.7747213021608985, -280.5281136083064553, -265.9823610640664242 ) ) ;
#66576=CARTESIAN_POINT ( 'NONE',  ( -85.69834922065264493, -280.4436098588087702, -215.2624740673053338 ) ) ;
#66577=CARTESIAN_POINT ( 'NONE',  ( -74.81667695509624139, -279.3041413628073428, -336.4640689456617224 ) ) ;
#66578=CONICAL_SURFACE ( 'NONE', #84667, 2.390969801828402019, 0.09862129276974965220 ) ;
#66579=CARTESIAN_POINT ( 'NONE',  ( -11.22657677776744833, -272.8784770234071857, -201.3956818251809864 ) ) ;
#66582=CARTESIAN_POINT ( 'NONE',  ( -87.53216568059616520, -279.4948925565139461, -217.2826061526542674 ) ) ;
#66583=CARTESIAN_POINT ( 'NONE',  ( 39.39242218108820026, -276.2933073416227217, -265.4399090191439541 ) ) ;
#66584=CARTESIAN_POINT ( 'NONE',  ( 37.70638377075786707, -277.5621275484356829, -271.1251693911075336 ) ) ;
#66585=CARTESIAN_POINT ( 'NONE',  ( -79.91308313417442832, -276.1901095226338612, -333.8778254082728267 ) ) ;
#66587=CARTESIAN_POINT ( 'NONE',  ( 3.672086032151444801, -284.4835922050748422, -333.6389085444195644 ) ) ;
#66588=CARTESIAN_POINT ( 'NONE',  ( -38.89077038600851211, -291.2293907658622061, -197.2160422166857927 ) ) ;
#66589=CARTESIAN_POINT ( 'NONE',  ( 36.59552054225849105, -286.6333361015286414, -249.0390530379026757 ) ) ;
#66590=CARTESIAN_POINT ( 'NONE',  ( -61.89169633937681425, -281.6153929035950227, -340.2382459872948175 ) ) ;
#66591=CARTESIAN_POINT ( 'NONE',  ( -94.75604204560765709, -282.4814043955014427, -316.4134227080695609 ) ) ;
#66592=CARTESIAN_POINT ( 'NONE',  ( -14.09351650650305920, -284.4357645358466016, -199.5904562764217474 ) ) ;
#66593=CARTESIAN_POINT ( 'NONE',  ( -66.24009643592751218, -280.8703140021155491, -202.8787943446638167 ) ) ;
#66595=CARTESIAN_POINT ( 'NONE',  ( -76.36589203693866068, -281.9642796306976038, -335.8711607248457085 ) ) ;
#66596=CARTESIAN_POINT ( 'NONE',  ( 31.58875881740157965, -295.9403147710103781, -300.0489787163130018 ) ) ;
#66597=CARTESIAN_POINT ( 'NONE',  ( -107.3309813039151095, -286.9099069751821389, -242.8054133358070885 ) ) ;
#66598=LINE ( 'NONE', #73251, #48914 ) ;
#66599=CARTESIAN_POINT ( 'NONE',  ( -66.48309816784104953, -293.5936382171083210, -200.6467498814550368 ) ) ;
#66600=CARTESIAN_POINT ( 'NONE',  ( -18.53949519698757697, -274.8097791831771133, -342.9660608962062156 ) ) ;
#66601=CARTESIAN_POINT ( 'NONE',  ( -40.34270959484315000, -288.2861179086589800, -347.1540703233896465 ) ) ;
#66602=CARTESIAN_POINT ( 'NONE',  ( 36.50841899612134966, -291.9575421380910143, -270.7846300421712158 ) ) ;
#66604=CARTESIAN_POINT ( 'NONE',  ( -94.84932671742315335, -276.5948735245735293, -316.1427413071419323 ) ) ;
#66605=CARTESIAN_POINT ( 'NONE',  ( -106.9560242299685910, -295.0315424710443040, -244.4309774975177731 ) ) ;
#66606=CARTESIAN_POINT ( 'NONE',  ( -63.98415273363372791, -290.7220956686800264, -338.9096281953815151 ) ) ;
#66608=CARTESIAN_POINT ( 'NONE',  ( 25.92596590112605170, -292.5992345257535021, -313.0215233704839761 ) ) ;
#66609=CARTESIAN_POINT ( 'NONE',  ( 27.74553075529512469, -289.6226049905581590, -305.2563260982196311 ) ) ;
#66610=CARTESIAN_POINT ( 'NONE',  ( -95.78493256127491406, -289.4539712661127737, -221.7780424918552455 ) ) ;
#66612=CARTESIAN_POINT ( 'NONE',  ( -1.918562638523249708, -287.9559594502072741, -205.8014211269785676 ) ) ;
#66614=CARTESIAN_POINT ( 'NONE',  ( 22.11685055905892838, -287.7594261060488634, -227.6461249135607829 ) ) ;
#66615=CARTESIAN_POINT ( 'NONE',  ( -85.32809321431076910, -297.6914147089660787, -328.4620033316837748 ) ) ;
#66616=CARTESIAN_POINT ( 'NONE',  ( 82.64890176555634582, -299.5541904835138780, -192.9651424135223863 ) ) ;
#66617=CARTESIAN_POINT ( 'NONE',  ( -70.45347019368922759, -290.6839807462974932, -339.4524373328906677 ) ) ;
#66618=CARTESIAN_POINT ( 'NONE',  ( -61.49601793128326932, -277.7601708064456147, -198.9269948074795309 ) ) ;
#66619=CARTESIAN_POINT ( 'NONE',  ( -97.03530360568313995, -278.2328109423121987, -318.9864700914941977 ) ) ;
#66620=CARTESIAN_POINT ( 'NONE',  ( -86.78789101243724247, -279.0531173677605352, -211.2931821224103714 ) ) ;
#66621=CARTESIAN_POINT ( 'NONE',  ( -75.72229887860241604, -283.5396852722327026, -205.9256441488438156 ) ) ;
#66622=CARTESIAN_POINT ( 'NONE',  ( -110.9948563253906997, -274.0459037229676369, -270.3801370180107710 ) ) ;
#66623=CARTESIAN_POINT ( 'NONE',  ( -3.768093034443908085, -278.6394812760652826, -204.1376373545090814 ) ) ;
#66624=CARTESIAN_POINT ( 'NONE',  ( -24.89133884712969191, -280.8933118828296074, -344.3732004978055556 ) ) ;
#66626=CARTESIAN_POINT ( 'NONE',  ( -112.0348454774373153, -277.2298124661746215, -254.6891549789921498 ) ) ;
#66627=CARTESIAN_POINT ( 'NONE',  ( -98.34171545634058020, -274.5460398394204731, -229.1074149326821896 ) ) ;
#66628=CARTESIAN_POINT ( 'NONE',  ( -114.0170112492860000, -283.5132591388492642, -267.1137264803851394 ) ) ;
#66629=CARTESIAN_POINT ( 'NONE',  ( -109.2904024274250645, -273.5331711080482364, -256.8239539616066054 ) ) ;
#66630=CARTESIAN_POINT ( 'NONE',  ( -99.10161077251049733, -274.5801524595136129, -225.2809147237078093 ) ) ;
#66631=CARTESIAN_POINT ( 'NONE',  ( 23.81352440969225981, -274.6661249362725812, -230.4596643937491649 ) ) ;
#66632=CARTESIAN_POINT ( 'NONE',  ( -61.63761508680422452, -297.3678486702981445, -341.3718377428374424 ) ) ;
#66633=CARTESIAN_POINT ( 'NONE',  ( -69.35536841980209033, -289.6285265735170924, -340.4049997764796558 ) ) ;
#66634=CARTESIAN_POINT ( 'NONE',  ( -79.09432247200943777, -277.5740299021042574, -207.3219212862858001 ) ) ;
#66635=CARTESIAN_POINT ( 'NONE',  ( -110.7824890474801549, -290.0927151617007098, -293.6751278584420675 ) ) ;
#66637=CARTESIAN_POINT ( 'NONE',  ( -98.31318920715831666, -289.0492812452019962, -310.9534737019613999 ) ) ;
#66638=CARTESIAN_POINT ( 'NONE',  ( -14.45196511547495000, -290.3485889822512718, -198.8848804238548098 ) ) ;
#66639=VERTEX_POINT ( 'NONE', #21165 ) ;
#66641=CARTESIAN_POINT ( 'NONE',  ( -107.7868233548885826, -289.8017717728951652, -289.9247424993363893 ) ) ;
#66644=CARTESIAN_POINT ( 'NONE',  ( 23.66711653063709520, -287.8700596135395813, -223.7483207976022754 ) ) ;
#66645=CARTESIAN_POINT ( 'NONE',  ( -82.08285599513421005, -292.1948066931273615, -326.5171145203363494 ) ) ;
#66646=CARTESIAN_POINT ( 'NONE',  ( 11.04069315161959963, -293.4602013878662774, -330.0279682166208772 ) ) ;
#66647=CARTESIAN_POINT ( 'NONE',  ( -65.05781846114622624, -284.7219546923205939, -341.6852220976551280 ) ) ;
#66648=CARTESIAN_POINT ( 'NONE',  ( -110.0959412061875895, -284.3065188182854968, -276.3461334077276774 ) ) ;
#66649=CARTESIAN_POINT ( 'NONE',  ( 29.52784386171970965, -276.4575154558016266, -239.7469643032682427 ) ) ;
#66650=CARTESIAN_POINT ( 'NONE',  ( 34.21288022044010546, -291.2950836534887458, -248.9274711602004970 ) ) ;
#66651=CARTESIAN_POINT ( 'NONE',  ( -5.119962510331440342, -273.2809468059714391, -204.4011015592346894 ) ) ;
#66654=CARTESIAN_POINT ( 'NONE',  ( 30.88164433630877426, -293.6790123540964146, -306.0166864331076226 ) ) ;
#66655=CARTESIAN_POINT ( 'NONE',  ( -75.47843760216241549, -287.4593674365907532, -206.4322242598769037 ) ) ;
#66656=CARTESIAN_POINT ( 'NONE',  ( -101.2995229053768895, -298.1909737508792091, -228.0182974826144289 ) ) ;
#66657=CARTESIAN_POINT ( 'NONE',  ( 32.36829771458664595, -287.9117171895986189, -248.3099355626429201 ) ) ;
#66658=CARTESIAN_POINT ( 'NONE',  ( -113.9976860803573118, -277.5596677635057290, -274.4452372310885835 ) ) ;
#66659=CARTESIAN_POINT ( 'NONE',  ( -36.38797637594077372, -292.7152250514493517, -193.4559499800649292 ) ) ;
#66660=CARTESIAN_POINT ( 'NONE',  ( 13.43689223911416164, -284.8930272069046055, -214.0604690638379566 ) ) ;
#66661=CARTESIAN_POINT ( 'NONE',  ( 30.88556681058348374, -294.3454674177526726, -306.0091801671821941 ) ) ;
#66662=CARTESIAN_POINT ( 'NONE',  ( -81.74526626170977295, -291.7619236875598290, -212.3280806636016393 ) ) ;
#66663=LINE ( 'NONE', #31610, #14657 ) ;
#66664=CARTESIAN_POINT ( 'NONE',  ( 180.0836269057152208, 251.0244910122962949, -164.3671539782268667 ) ) ;
#66665=CARTESIAN_POINT ( 'NONE',  ( -112.4510006355684908, -285.8986872631709275, -284.1156267515526110 ) ) ;
#66666=CARTESIAN_POINT ( 'NONE',  ( 25.18497378105905682, -279.6952119285918457, -320.2651865833026363 ) ) ;
#66668=CARTESIAN_POINT ( 'NONE',  ( -5.912845675140160573, -281.5493938731575554, -336.6052296906557331 ) ) ;
#66669=CARTESIAN_POINT ( 'NONE',  ( -111.4213247328650880, -277.9565197447284959, -291.2884567999438445 ) ) ;
#66670=CARTESIAN_POINT ( 'NONE',  ( 21.64133933810120780, -284.1855163729746323, -316.4157538635529932 ) ) ;
#66671=CARTESIAN_POINT ( 'NONE',  ( -61.35559941387249694, -183.8768497150109340, -360.9409086351379869 ) ) ;
#66672=CARTESIAN_POINT ( 'NONE',  ( -99.32126633906587188, -282.5287862902465008, -315.1389364568215683 ) ) ;
#66673=CARTESIAN_POINT ( 'NONE',  ( 33.84973376563834790, -285.2808363263382603, -247.8766542323534736 ) ) ;
#66674=CARTESIAN_POINT ( 'NONE',  ( -68.36039097110868568, -275.5094503813119218, -201.2228144700276573 ) ) ;
#66675=CARTESIAN_POINT ( 'NONE',  ( -104.8214434374840778, -297.4197765858179991, -242.3526784617394867 ) ) ;
#66677=CARTESIAN_POINT ( 'NONE',  ( -10.32418687202441809, -293.3768298803088328, -338.7080085908231126 ) ) ;
#66678=CARTESIAN_POINT ( 'NONE',  ( -109.6380863644192942, -278.8704263816352409, -296.7188510151196965 ) ) ;
#66679=CARTESIAN_POINT ( 'NONE',  ( -56.60017204741144070, -277.3072711218024438, -340.8274729419055689 ) ) ;
#66680=CARTESIAN_POINT ( 'NONE',  ( -107.7989798829545407, -274.0206871230410570, -239.9403905836601041 ) ) ;
#66681=CARTESIAN_POINT ( 'NONE',  ( -84.68639591732380723, -276.6072652499581181, -330.7607884625851398 ) ) ;
#66683=CARTESIAN_POINT ( 'NONE',  ( -5.654136641094509308, -274.6353443764088524, -338.3521506364288030 ) ) ;
#66685=CARTESIAN_POINT ( 'NONE',  ( -96.04698207720574032, -297.3142253595705142, -319.2925613599231269 ) ) ;
#66687=CARTESIAN_POINT ( 'NONE',  ( 26.40820234725076787, -24.66803830325296687, -341.1985388896944755 ) ) ;
#66688=CARTESIAN_POINT ( 'NONE',  ( -53.74551868804229571, -284.3471893230417322, -341.8636884958267501 ) ) ;
#66689=CARTESIAN_POINT ( 'NONE',  ( -60.89598388462611211, -285.1137155922242528, -342.6598846594791894 ) ) ;
#66690=CARTESIAN_POINT ( 'NONE',  ( -54.77261557253265067, -285.1708422916265135, -199.3153977015881537 ) ) ;
#66691=CARTESIAN_POINT ( 'NONE',  ( -109.0623672766620729, -277.1790428158155351, -252.9661094684980753 ) ) ;
#66692=CARTESIAN_POINT ( 'NONE',  ( -106.3536204270571375, -286.0511008532281494, -297.8545499948111797 ) ) ;
#66693=CARTESIAN_POINT ( 'NONE',  ( -89.95515244568397861, -277.7726323302619562, -218.6890878146726322 ) ) ;
#66694=CARTESIAN_POINT ( 'NONE',  ( -11.13073371842595627, -277.7819877096691243, -338.8243293707045041 ) ) ;
#66696=CARTESIAN_POINT ( 'NONE',  ( -54.23184288650222129, -274.3216581455266692, -199.2786903435467707 ) ) ;
#66697=CARTESIAN_POINT ( 'NONE',  ( 36.32680637813746216, -282.6316718168910143, -292.3870917561814053 ) ) ;
#66698=CARTESIAN_POINT ( 'NONE',  ( 0.8432681186432263720, -283.0493417035392554, -337.1703136565325849 ) ) ;
#66702=CARTESIAN_POINT ( 'NONE',  ( 32.90612757349362028, -289.7803605344437869, -298.8831495163289560 ) ) ;
#66703=CARTESIAN_POINT ( 'NONE',  ( -100.0298913023517429, -296.2683635824841986, -232.5426995085460646 ) ) ;
#66704=CARTESIAN_POINT ( 'NONE',  ( 15.37433248308129308, -292.1220328462279667, -214.3028865048143814 ) ) ;
#66705=CARTESIAN_POINT ( 'NONE',  ( 18.33677346312641987, -286.7142773349410731, -318.7139422826398913 ) ) ;
#66706=CARTESIAN_POINT ( 'NONE',  ( -34.57387675725116338, -287.5915584499234114, -343.9482619998299242 ) ) ;
#66707=CARTESIAN_POINT ( 'NONE',  ( 18.95650955822851458, -288.0921982289884227, -223.2496955252817088 ) ) ;
#66708=CARTESIAN_POINT ( 'NONE',  ( -93.72452607665498192, -275.8649272248415514, -319.8179434850908365 ) ) ;
#66709=CARTESIAN_POINT ( 'NONE',  ( -15.20433921795632592, -287.1701872580026134, -343.3297796228917491 ) ) ;
#66710=CARTESIAN_POINT ( 'NONE',  ( -40.75171745722013128, -288.0095491815368973, -195.3878388967245598 ) ) ;
#66711=CARTESIAN_POINT ( 'NONE',  ( -23.67098173512307824, -286.8778148181965548, -344.3269977883953175 ) ) ;
#66713=CARTESIAN_POINT ( 'NONE',  ( 7.948848076696403808, -283.3573060838906486, -327.9773882919641323 ) ) ;
#66714=CARTESIAN_POINT ( 'NONE',  ( -73.81221612591677683, -293.5691591439108947, -204.6349444228563357 ) ) ;
#66717=CARTESIAN_POINT ( 'NONE',  ( -92.62617576607279091, -299.1884703524148108, -218.7780632528977662 ) ) ;
#66718=CARTESIAN_POINT ( 'NONE',  ( -51.84940131230460736, -279.0590405015331612, -198.6006392681399291 ) ) ;
#66719=CARTESIAN_POINT ( 'NONE',  ( 9.010565118092618064, -280.4163668864175634, -329.3890097020399139 ) ) ;
#66720=CARTESIAN_POINT ( 'NONE',  ( 25.57654286247664643, -293.3340608566641663, -314.4913720465977462 ) ) ;
#66721=CARTESIAN_POINT ( 'NONE',  ( -60.75055225159313466, -296.1433127619204129, -200.3180259472798070 ) ) ;
#66722=CARTESIAN_POINT ( 'NONE',  ( 16.62533118532242682, -274.3568591648520396, -321.6336616008841247 ) ) ;
#66723=CARTESIAN_POINT ( 'NONE',  ( -84.78376024725687898, -297.0371047690934461, -326.5571878338938632 ) ) ;
#66725=CARTESIAN_POINT ( 'NONE',  ( -78.50871170176674241, -272.0842206655200926, -205.9881154884022010 ) ) ;
#66726=CARTESIAN_POINT ( 'NONE',  ( -111.8901102181933567, -294.9793387879476541, -255.5800720510984547 ) ) ;
#66727=CARTESIAN_POINT ( 'NONE',  ( 21.81083818433715393, -295.5862676791116996, -314.1372773570800518 ) ) ;
#66729=CARTESIAN_POINT ( 'NONE',  ( -3.059060201505739318, -295.3897480925137415, -334.9931713849321113 ) ) ;
#66731=CARTESIAN_POINT ( 'NONE',  ( -75.25685377393928377, -283.5699375086498435, -205.1792469172315236 ) ) ;
#66732=CARTESIAN_POINT ( 'NONE',  ( -96.40841390429547175, -295.9515655637036389, -313.2791125579200298 ) ) ;
#66733=CARTESIAN_POINT ( 'NONE',  ( -99.78847660527259222, -283.9538283504805349, -315.4990862996025385 ) ) ;
#66734=CARTESIAN_POINT ( 'NONE',  ( -34.00381809868024874, -282.0139860387562294, -194.8748759016867211 ) ) ;
#66735=CARTESIAN_POINT ( 'NONE',  ( -2.228762407993491124, -286.1707241459696434, -201.8421655686406666 ) ) ;
#66736=CARTESIAN_POINT ( 'NONE',  ( -63.41624496468342898, -289.7114337277871527, -200.2173617543675732 ) ) ;
#66738=CARTESIAN_POINT ( 'NONE',  ( -37.30987171927208834, -271.5523547857346784, -195.3611179825600175 ) ) ;
#66739=CARTESIAN_POINT ( 'NONE',  ( -17.01954791531377609, -285.0047789399824296, -199.6803399071605440 ) ) ;
#66740=CARTESIAN_POINT ( 'NONE',  ( -111.2477783009753836, -289.2148846050994280, -290.8399880543827862 ) ) ;
#66742=CARTESIAN_POINT ( 'NONE',  ( -110.5323212056413240, -298.2808308655049814, -260.5099338820116941 ) ) ;
#66743=CARTESIAN_POINT ( 'NONE',  ( -107.0311960033911873, -279.5726451904997134, -301.8263652807584663 ) ) ;
#66744=CARTESIAN_POINT ( 'NONE',  ( 28.13278233394262173, -292.0684992701981741, -307.7692669019813820 ) ) ;
#66745=CARTESIAN_POINT ( 'NONE',  ( 7.158569387886407398, -280.3439879132166084, -212.4022905858366812 ) ) ;
#66746=CARTESIAN_POINT ( 'NONE',  ( -39.10571175695683621, -295.2403958382071778, -347.3409092754811240 ) ) ;
#66747=CARTESIAN_POINT ( 'NONE',  ( -37.94592848949424280, -284.1244890159491661, -194.8035299426656195 ) ) ;
#66748=CARTESIAN_POINT ( 'NONE',  ( -107.7380240075472244, -280.8897397479200890, -244.3390825784085791 ) ) ;
#66749=CARTESIAN_POINT ( 'NONE',  ( -4.241001199789314668, -293.6634512845080280, -335.7031955238873024 ) ) ;
#66750=CARTESIAN_POINT ( 'NONE',  ( -109.2750270191963580, -270.8344936132971270, -248.3745720545137772 ) ) ;
#66753=CARTESIAN_POINT ( 'NONE',  ( 30.45628928834290861, -283.1185492304643958, -239.0078743276770865 ) ) ;
#66754=CARTESIAN_POINT ( 'NONE',  ( -72.15942204334145060, -295.0334859749779639, -334.6071260114547385 ) ) ;
#66756=CARTESIAN_POINT ( 'NONE',  ( -54.49178911615187104, -280.7666405000204009, -345.3538533559490702 ) ) ;
#66757=CARTESIAN_POINT ( 'NONE',  ( -63.49251044722220882, -272.9170078647272817, -198.1095163396097973 ) ) ;
#66758=CARTESIAN_POINT ( 'NONE',  ( 27.03893497890713959, -289.4141400277896992, -311.7920166814591312 ) ) ;
#66759=CARTESIAN_POINT ( 'NONE',  ( -74.97778835006916154, -291.3694006683082875, -207.7519247701086442 ) ) ;
#66760=CARTESIAN_POINT ( 'NONE',  ( -32.94076872930077116, -281.6287284087828766, -196.7993102558860983 ) ) ;
#66761=CARTESIAN_POINT ( 'NONE',  ( -89.82526302268895790, -274.8961100652074379, -218.4774400045996003 ) ) ;
#66762=CARTESIAN_POINT ( 'NONE',  ( -38.34393925807676595, -278.8342387412107541, -196.9584190451636232 ) ) ;
#66763=CARTESIAN_POINT ( 'NONE',  ( 25.67839293862412120, -278.1013100876400586, -311.1197902605612740 ) ) ;
#66765=CARTESIAN_POINT ( 'NONE',  ( 21.85221839399833499, -274.7231276717928949, -221.1160165558101767 ) ) ;
#66766=CARTESIAN_POINT ( 'NONE',  ( 13.87657676184798738, -294.6974971904480185, -216.3425812706616682 ) ) ;
#66769=CARTESIAN_POINT ( 'NONE',  ( 35.89480652357097057, -291.4442121337436333, -250.9017380571721958 ) ) ;
#66770=CARTESIAN_POINT ( 'NONE',  ( -63.08294680178118341, -297.3743099841260005, -201.9740623292235284 ) ) ;
#66773=CARTESIAN_POINT ( 'NONE',  ( -42.03087026812858085, -293.5141712697696335, -194.1986637375347584 ) ) ;
#66774=CARTESIAN_POINT ( 'NONE',  ( 10.59707575819634329, -277.1948066931274184, -210.1954327657594490 ) ) ;
#66775=CARTESIAN_POINT ( 'NONE',  ( 34.42101848358568361, -289.2779139193150399, -249.0994495047464170 ) ) ;
#66776=CARTESIAN_POINT ( 'NONE',  ( 12.96170564915455792, -274.3481182168935106, -325.8353443617008907 ) ) ;
#66777=CARTESIAN_POINT ( 'NONE',  ( 29.13651351811480694, -277.0264742199000239, -236.8654271353415766 ) ) ;
#66779=CARTESIAN_POINT ( 'NONE',  ( -30.65371873581474915, -290.2172107132033148, -196.2221599197860087 ) ) ;
#66780=CARTESIAN_POINT ( 'NONE',  ( -88.12141876326258227, -281.2106996960274614, -214.1318937876493749 ) ) ;
#66782=CARTESIAN_POINT ( 'NONE',  ( -8.461594524924265670, -282.0123982166359156, -337.5164019799333914 ) ) ;
#66783=CARTESIAN_POINT ( 'NONE',  ( -112.4177867730260800, -279.8291844199134744, -254.6429016545420154 ) ) ;
#66784=CARTESIAN_POINT ( 'NONE',  ( -50.04286232407507384, -282.0055599113663334, -345.9573482249328436 ) ) ;
#66785=CARTESIAN_POINT ( 'NONE',  ( -77.68102657602891270, -278.5205858967833024, -335.7341309429302783 ) ) ;
#66786=CARTESIAN_POINT ( 'NONE',  ( 28.50749117222059681, -277.5786736424022365, -308.9174631994290507 ) ) ;
#66787=CARTESIAN_POINT ( 'NONE',  ( 7.399455738971494334, -283.1948066931273615, -214.2051214447836571 ) ) ;
#66789=CARTESIAN_POINT ( 'NONE',  ( -104.5493569401108829, -298.1117102138980499, -303.7670087738766256 ) ) ;
#66790=CARTESIAN_POINT ( 'NONE',  ( -82.72691286868111149, -290.7692845221287712, -327.9320180720994244 ) ) ;
#66791=CARTESIAN_POINT ( 'NONE',  ( -107.8254883898565879, -276.2507622517907748, -295.0920485928824064 ) ) ;
#66792=CARTESIAN_POINT ( 'NONE',  ( -38.87693049490011532, -290.8312997388157441, -346.3322775390297465 ) ) ;
#66793=CARTESIAN_POINT ( 'NONE',  ( -93.51284384142114448, -290.5637697198045544, -223.5580854985755650 ) ) ;
#66794=CARTESIAN_POINT ( 'NONE',  ( -5.657569261768225388, -288.1541658785433242, -340.4727629119571475 ) ) ;
#66796=CARTESIAN_POINT ( 'NONE',  ( -102.4868907441952928, -282.4833049739951889, -305.1476620427841908 ) ) ;
#66797=CARTESIAN_POINT ( 'NONE',  ( -97.54672305710471392, -291.8152614121597708, -313.7917603447917827 ) ) ;
#66798=CARTESIAN_POINT ( 'NONE',  ( -106.8339590332081457, -282.7069109963416054, -295.0393749829704007 ) ) ;
#66799=CARTESIAN_POINT ( 'NONE',  ( 36.19649311150399740, -282.8796814814920140, -271.3034798066948383 ) ) ;
#66800=CARTESIAN_POINT ( 'NONE',  ( -36.07865563205614023, -289.9779596449803307, -347.1285035105844372 ) ) ;
#66801=CARTESIAN_POINT ( 'NONE',  ( -107.1735840877335590, -278.7581654899304340, -292.0129478101076757 ) ) ;
#66802=CARTESIAN_POINT ( 'NONE',  ( 3.940539295488321159, -291.3894212940592752, -205.7708353016273293 ) ) ;
#66803=CARTESIAN_POINT ( 'NONE',  ( 32.56086856997399792, -287.9448447371245834, -238.3302530837080155 ) ) ;
#66804=CARTESIAN_POINT ( 'NONE',  ( -8.250585376719735464, -289.1736423544753052, -341.6020112660514769 ) ) ;
#66805=CARTESIAN_POINT ( 'NONE',  ( -108.0927015866721490, -284.4815127564268096, -288.3415461514354661 ) ) ;
#66808=CARTESIAN_POINT ( 'NONE',  ( -53.15501775893466174, -293.7120492957038209, -196.2113074505303132 ) ) ;
#66809=CARTESIAN_POINT ( 'NONE',  ( 35.01451407175223807, -292.5541256450414380, -295.3804821535210863 ) ) ;
#66810=CARTESIAN_POINT ( 'NONE',  ( -29.70075624538922909, -276.0119215304806630, -343.2477860638952052 ) ) ;
#66811=CARTESIAN_POINT ( 'NONE',  ( -101.4601106621486224, -296.4601683663465224, -227.8854986308761283 ) ) ;
#66812=CARTESIAN_POINT ( 'NONE',  ( 13.39438997519455121, -291.2577753230997359, -216.9143508928158894 ) ) ;
#66813=CARTESIAN_POINT ( 'NONE',  ( -58.16875831301216238, -296.0191570815654813, -199.3385324285015088 ) ) ;
#66814=CARTESIAN_POINT ( 'NONE',  ( -94.61031751668357970, -292.4026886597474117, -224.4343232609355709 ) ) ;
#66815=CARTESIAN_POINT ( 'NONE',  ( 19.94389446515256026, -295.2754580729890677, -316.1259345595842660 ) ) ;
#66816=CARTESIAN_POINT ( 'NONE',  ( -25.22895927321087228, -292.8980477503152429, -344.5981907666093207 ) ) ;
#66817=CARTESIAN_POINT ( 'NONE',  ( 60.19128830256915563, -301.2732859087743691, -195.3278605009263060 ) ) ;
#66818=CARTESIAN_POINT ( 'NONE',  ( 25.90528312414506118, -288.9997458554204854, -307.3833121448694214 ) ) ;
#66819=CARTESIAN_POINT ( 'NONE',  ( 22.23351816859807428, -278.1618069544609853, -316.5253106550804887 ) ) ;
#66820=CARTESIAN_POINT ( 'NONE',  ( -112.5085079222426003, -277.4173112377816892, -256.0345818978447028 ) ) ;
#66821=CARTESIAN_POINT ( 'NONE',  ( -76.37382014607375424, -272.8935266381818110, -204.0439799770036586 ) ) ;
#66822=CARTESIAN_POINT ( 'NONE',  ( 4.173423967329497941, -280.5681187145156059, -332.2118747651024933 ) ) ;
#66823=CARTESIAN_POINT ( 'NONE',  ( -111.4025260527821501, -276.7247644265662530, -288.3444230124958381 ) ) ;
#66824=CARTESIAN_POINT ( 'NONE',  ( -108.6493845057013488, -295.4707646075503362, -252.5203891492550667 ) ) ;
#66825=CARTESIAN_POINT ( 'NONE',  ( -94.72225332419415622, -275.2202216751836659, -222.0458084243138330 ) ) ;
#66826=CARTESIAN_POINT ( 'NONE',  ( 11.60863304955299213, -275.4040876644211266, -215.9997109070220063 ) ) ;
#66829=CARTESIAN_POINT ( 'NONE',  ( -108.8616546510138221, -288.8794171114324172, -246.4639909370486066 ) ) ;
#66831=CARTESIAN_POINT ( 'NONE',  ( -57.29089898836343053, -289.3025524128559596, -344.7871143467750130 ) ) ;
#66832=CARTESIAN_POINT ( 'NONE',  ( 0.2558075010870646260, -276.5517316177546832, -205.2581371564674555 ) ) ;
#66833=CARTESIAN_POINT ( 'NONE',  ( -110.3868204106277204, -294.3427326982731529, -286.6226933687775613 ) ) ;
#66835=CARTESIAN_POINT ( 'NONE',  ( -1.718098331928909372, -281.7894003285283020, -338.4428175501761302 ) ) ;
#66839=CARTESIAN_POINT ( 'NONE',  ( 19.42697874413789449, -280.2317892636173156, -319.3938110875790812 ) ) ;
#66841=CARTESIAN_POINT ( 'NONE',  ( -57.75071423307057472, -290.5777154140786251, -199.8054558447315969 ) ) ;
#66842=CARTESIAN_POINT ( 'NONE',  ( -57.71094265623317199, -283.9260509383547628, -198.9216310065164066 ) ) ;
#66845=CARTESIAN_POINT ( 'NONE',  ( 37.64040703607278715, -291.5935751674341532, -273.6000701297232354 ) ) ;
#66846=CARTESIAN_POINT ( 'NONE',  ( -54.11617747601757600, -278.8711408014724498, -342.2821602979754516 ) ) ;
#66847=CARTESIAN_POINT ( 'NONE',  ( -33.06549193672525178, -284.2045168166098961, -346.8576654642611174 ) ) ;
#66848=CARTESIAN_POINT ( 'NONE',  ( 13.02320048660527974, -272.8285620592045575, -213.9645318959786948 ) ) ;
#66849=CARTESIAN_POINT ( 'NONE',  ( -87.69450223319059035, -285.3246945150340821, -217.5066449441906968 ) ) ;
#66850=CARTESIAN_POINT ( 'NONE',  ( 3.475893269915882211, -277.9165547436763291, -331.5926375238618107 ) ) ;
#66851=CARTESIAN_POINT ( 'NONE',  ( 20.97180314478336172, -276.9744973678308497, -314.5441131671724406 ) ) ;
#66852=CARTESIAN_POINT ( 'NONE',  ( -70.21325028285555447, -287.6191410338793162, -202.9484942099033162 ) ) ;
#66854=FACE_OUTER_BOUND ( 'NONE', #39932, .T. ) ;
#66855=CARTESIAN_POINT ( 'NONE',  ( -97.40877091635981344, -295.7397667153531415, -318.5581936505013800 ) ) ;
#66856=CARTESIAN_POINT ( 'NONE',  ( -42.81943693280844343, -287.9626094766422852, -195.9046641415179124 ) ) ;
#66858=CARTESIAN_POINT ( 'NONE',  ( -19.05039376806006857, -289.7666405000204009, -190.3683826091709363 ) ) ;
#66859=CARTESIAN_POINT ( 'NONE',  ( -108.2217078181806329, -277.8461775948298964, -241.0777264638954875 ) ) ;
#66860=CARTESIAN_POINT ( 'NONE',  ( -74.27313864602086824, -289.9694517170592576, -203.7089667408608591 ) ) ;
#66861=CARTESIAN_POINT ( 'NONE',  ( -42.74409273166229184, -287.5029134548743173, -196.8533256199991115 ) ) ;
#66862=CARTESIAN_POINT ( 'NONE',  ( -110.4901901947326905, -280.1655134037587231, -281.6426256381563462 ) ) ;
#66863=CARTESIAN_POINT ( 'NONE',  ( 26.63442371319922941, -288.4242674244037516, -228.5799993914037316 ) ) ;
#66864=CARTESIAN_POINT ( 'NONE',  ( -26.42722136458372972, -284.9135586049499693, -344.6154075554599672 ) ) ;
#66865=CARTESIAN_POINT ( 'NONE',  ( 22.64233765057464609, -276.3660845546355631, -318.6615273389513163 ) ) ;
#66866=CARTESIAN_POINT ( 'NONE',  ( -52.95506504555213922, -295.8712886083820308, -197.3144395312322104 ) ) ;
#66867=CARTESIAN_POINT ( 'NONE',  ( -56.55460229822654128, -279.6445882519741417, -195.7416199393135230 ) ) ;
#66868=CARTESIAN_POINT ( 'NONE',  ( -109.8857681398556423, -298.6882604995303723, -253.6676342733145759 ) ) ;
#66870=CARTESIAN_POINT ( 'NONE',  ( 39.58706461736021254, -278.0519495502701943, -270.3284710469133074 ) ) ;
#66871=CARTESIAN_POINT ( 'NONE',  ( -35.52524190666022008, -272.3144843020784833, -194.3832051352771657 ) ) ;
#66873=CARTESIAN_POINT ( 'NONE',  ( 151.9709352735115147, -299.5541904835127980, -195.3611179825600175 ) ) ;
#66874=CARTESIAN_POINT ( 'NONE',  ( -85.15024169605698035, -277.2407497297832606, -325.6760518972466798 ) ) ;
#66875=CARTESIAN_POINT ( 'NONE',  ( -60.76438287097140289, -274.9600488305526369, -197.3716450990360727 ) ) ;
#66876=CARTESIAN_POINT ( 'NONE',  ( 0.7411836450362718764, -281.6159739079147357, -337.0284904910478758 ) ) ;
#66877=CARTESIAN_POINT ( 'NONE',  ( -2.874775822079837617, -290.3505950851243824, -335.9160213339897609 ) ) ;
#66878=CARTESIAN_POINT ( 'NONE',  ( -84.80046405501836659, -298.9313138850195060, -210.6085157178228826 ) ) ;
#66879=CARTESIAN_POINT ( 'NONE',  ( -97.92940309623408268, -298.3864361357140069, -223.4662933586699296 ) ) ;
#66880=CARTESIAN_POINT ( 'NONE',  ( -37.58074946566359387, -294.0493461499370937, -195.5154062998323354 ) ) ;
#66881=CARTESIAN_POINT ( 'NONE',  ( 22.46000633220254983, -280.1684892219421954, -315.3687749933597502 ) ) ;
#66882=CARTESIAN_POINT ( 'NONE',  ( 23.27210241904560561, -282.8803055347647728, -227.1490694301642179 ) ) ;
#66883=CARTESIAN_POINT ( 'NONE',  ( -3.333295855144573050, -272.5235449935348697, -203.8992293558194433 ) ) ;
#66884=CARTESIAN_POINT ( 'NONE',  ( -100.7420801062649787, -285.5889673348611382, -312.7266960608000659 ) ) ;
#66885=CARTESIAN_POINT ( 'NONE',  ( -39.98294687965398708, -288.0063123397029017, -343.6724244598802329 ) ) ;
#66886=CARTESIAN_POINT ( 'NONE',  ( 155.1585690732346450, 206.2207167234212193, -217.1754125233248374 ) ) ;
#66888=CARTESIAN_POINT ( 'NONE',  ( -31.88710179228944952, -287.5594633726584561, -346.6291079395904262 ) ) ;
#66889=CARTESIAN_POINT ( 'NONE',  ( 3.622960444184753381, -288.1511743511123314, -330.8702800020743666 ) ) ;
#66891=CARTESIAN_POINT ( 'NONE',  ( -16.21374430696123881, -283.8650357875006307, -344.1393293041872425 ) ) ;
#66892=CARTESIAN_POINT ( 'NONE',  ( 30.29921685870103332, -276.2554330213101821, -298.0055659719299683 ) ) ;
#66893=CARTESIAN_POINT ( 'NONE',  ( -58.83881269432927041, -290.7007250168816768, -196.7447702036221813 ) ) ;
#66894=CARTESIAN_POINT ( 'NONE',  ( 38.69266256807665627, -282.0553151159350023, -258.5230288893407646 ) ) ;
#66895=CARTESIAN_POINT ( 'NONE',  ( 18.63824324903709950, -282.3594468031603810, -218.5059958408970715 ) ) ;
#66896=CARTESIAN_POINT ( 'NONE',  ( -97.15328148535061814, -284.2350876661647021, -318.8412887183046109 ) ) ;
#66897=CARTESIAN_POINT ( 'NONE',  ( -30.26238517892669577, -280.1440608554726737, -197.6548388104711478 ) ) ;
#66898=CARTESIAN_POINT ( 'NONE',  ( -53.35057174420112602, -292.7666405000204577, -340.3538533559490702 ) ) ;
#66899=CARTESIAN_POINT ( 'NONE',  ( -113.6817389704806232, -274.0367189774781309, -270.3800200741469553 ) ) ;
#66902=CARTESIAN_POINT ( 'NONE',  ( 37.53361432508727802, -277.5681354020764502, -271.5902829283072037 ) ) ;
#66903=CARTESIAN_POINT ( 'NONE',  ( -84.83675082977744353, -218.8559137767458367, -351.9183727634863885 ) ) ;
#66905=CARTESIAN_POINT ( 'NONE',  ( -55.31070341228750920, -297.1635380649868807, -199.4496675265181693 ) ) ;
#66906=CARTESIAN_POINT ( 'NONE',  ( 38.75475483610038197, -293.2018864487969836, -281.7126132640497644 ) ) ;
#66907=CARTESIAN_POINT ( 'NONE',  ( -81.97344496812658576, -219.2901136445231316, -349.2013451768860364 ) ) ;
#66908=CIRCLE ( 'NONE', #86561, 2.500000000000008882 ) ;
#66909=CARTESIAN_POINT ( 'NONE',  ( -70.45713483483130801, -296.1988329782084861, -201.4991235301377799 ) ) ;
#66910=CARTESIAN_POINT ( 'NONE',  ( -13.04349295403358866, -287.1309604114507010, -340.0463929163666990 ) ) ;
#66911=CARTESIAN_POINT ( 'NONE',  ( -99.75924385471867595, -297.8645385357791042, -310.6412569139009747 ) ) ;
#66912=CARTESIAN_POINT ( 'NONE',  ( 17.24575557252470759, -288.1672371298577104, -221.1340723638584507 ) ) ;
#66914=CARTESIAN_POINT ( 'NONE',  ( -36.26568712721649490, -295.9802549357141288, -347.1313467208539691 ) ) ;
#66915=AXIS2_PLACEMENT_3D ( 'NONE', #30583, #88793, #59484 ) ;
#66916=CARTESIAN_POINT ( 'NONE',  ( -108.7263763185654284, -285.2504037482521539, -254.7393821814821138 ) ) ;
#66917=CARTESIAN_POINT ( 'NONE',  ( -60.01583976572951684, -296.5597358308956473, -197.1355909887807059 ) ) ;
#66918=CARTESIAN_POINT ( 'NONE',  ( -0.8894949029108201177, -293.3264616937420328, -202.7194477265767887 ) ) ;
#66919=CARTESIAN_POINT ( 'NONE',  ( 39.59422962047796801, -294.0078450261160583, -267.4326853852362547 ) ) ;
#66920=CARTESIAN_POINT ( 'NONE',  ( -106.5719643720372716, -291.0263627114725864, -247.2057618589018944 ) ) ;
#66923=CARTESIAN_POINT ( 'NONE',  ( -112.9017001288127346, -274.4719972107771468, -270.3855110958305090 ) ) ;
#66924=CARTESIAN_POINT ( 'NONE',  ( 26.60757217046068845, -273.7896616436511863, -228.1888606222470059 ) ) ;
#66926=CARTESIAN_POINT ( 'NONE',  ( -45.64920957719182582, -276.6622845402636699, -346.9027751304702178 ) ) ;
#66927=CARTESIAN_POINT ( 'NONE',  ( -79.29326907088395160, -271.8756530370084192, -209.5824471396249180 ) ) ;
#66928=CARTESIAN_POINT ( 'NONE',  ( -109.6847239637551041, -280.1958005568909016, -287.0712763307971613 ) ) ;
#66929=CARTESIAN_POINT ( 'NONE',  ( -5.772504451945826176, -274.7721814257769779, -337.5632956575348089 ) ) ;
#66930=CARTESIAN_POINT ( 'NONE',  ( -63.23383045339200947, -298.9124187889054269, -201.6289025273190703 ) ) ;
#66931=CARTESIAN_POINT ( 'NONE',  ( -89.41788040884343047, -274.2373398920433942, -218.8685952697086634 ) ) ;
#66932=CARTESIAN_POINT ( 'NONE',  ( -108.2294805023921498, -274.6651982674780470, -242.8501941320334652 ) ) ;
#66933=CARTESIAN_POINT ( 'NONE',  ( -8.300646040271290715, -272.4504779498249150, -200.7713833410523137 ) ) ;
#66934=CARTESIAN_POINT ( 'NONE',  ( 18.05509406843059494, -294.8820821946591764, -318.0780878978462169 ) ) ;
#66935=CARTESIAN_POINT ( 'NONE',  ( -66.78328110061660539, -290.2333653970372893, -202.9180440001503314 ) ) ;
#66937=CARTESIAN_POINT ( 'NONE',  ( -2.747158939369240827, -277.0995192502858231, -339.0980127403515212 ) ) ;
#66938=CARTESIAN_POINT ( 'NONE',  ( -16.64269548449760805, -274.4936814796191697, -200.3044730340681099 ) ) ;
#66939=CARTESIAN_POINT ( 'NONE',  ( -102.5068597461124966, -282.7097126234372695, -310.4460309048053546 ) ) ;
#66940=CARTESIAN_POINT ( 'NONE',  ( -110.8140545556915839, -298.7563420454741276, -254.4314279822453386 ) ) ;
#66942=CARTESIAN_POINT ( 'NONE',  ( -54.78495104298879426, -285.0194472865028956, -199.2570719344716110 ) ) ;
#66943=CARTESIAN_POINT ( 'NONE',  ( -104.1662447159930878, -282.0962989774749303, -304.8914503707903236 ) ) ;
#66945=CARTESIAN_POINT ( 'NONE',  ( -96.92188341286590969, -276.1847858055671736, -314.2933678676043883 ) ) ;
#66946=CARTESIAN_POINT ( 'NONE',  ( -64.56789046347860506, -275.9892728393234620, -338.7826994224380428 ) ) ;
#66947=CARTESIAN_POINT ( 'NONE',  ( 33.90511230064365833, -283.2477437889155567, -246.7694381402021691 ) ) ;
#66948=CARTESIAN_POINT ( 'NONE',  ( 35.77230737555238704, -276.6654787420447974, -263.3677301236903645 ) ) ;
#66950=CARTESIAN_POINT ( 'NONE',  ( -0.4150895636654400311, -272.9344185597497585, -203.6914525832594620 ) ) ;
#66951=CARTESIAN_POINT ( 'NONE',  ( 9.656385950408930441, -282.6968129654923132, -211.6326093896558120 ) ) ;
#66954=CARTESIAN_POINT ( 'NONE',  ( 23.52844107698648557, -288.8662780168637596, -225.5934945264107228 ) ) ;
#66956=CARTESIAN_POINT ( 'NONE',  ( -92.28431649405821702, -287.8371035508541809, -321.4873099704672086 ) ) ;
#66958=CARTESIAN_POINT ( 'NONE',  ( -71.83812560875631448, -296.3804402151587283, -205.5616057012519491 ) ) ;
#66959=CARTESIAN_POINT ( 'NONE',  ( -100.7546451304853576, -289.2144811071910340, -231.7649538593386183 ) ) ;
#66960=CARTESIAN_POINT ( 'NONE',  ( -51.00049622308160480, -154.6998088915060237, -359.8797964913271130 ) ) ;
#66961=CARTESIAN_POINT ( 'NONE',  ( -44.74174808262339553, -295.9584584443144308, -195.6753159266001205 ) ) ;
#66962=CARTESIAN_POINT ( 'NONE',  ( 32.22478160262502911, -286.4362108120465109, -301.7173353969674849 ) ) ;
#66963=CARTESIAN_POINT ( 'NONE',  ( -15.88060979045458154, -284.3700096286873418, -340.9717546821901237 ) ) ;
#66964=CARTESIAN_POINT ( 'NONE',  ( -109.0139266078943479, -283.1146767995436448, -245.1209522924006592 ) ) ;
#66965=CARTESIAN_POINT ( 'NONE',  ( -90.75918558089340138, -291.2677466969161628, -220.5875131363787318 ) ) ;
#66966=CARTESIAN_POINT ( 'NONE',  ( 34.51970584627218841, -283.1848775805641480, -286.2139805139627811 ) ) ;
#66967=CARTESIAN_POINT ( 'NONE',  ( 32.88673142598792509, -282.0842894519435049, -249.8533358341228450 ) ) ;
#66968=CARTESIAN_POINT ( 'NONE',  ( -97.69629866007362295, -291.9183837106073156, -315.5015036296520634 ) ) ;
#66970=CARTESIAN_POINT ( 'NONE',  ( -60.15011439280849714, -297.9312707115456078, -196.7612125331842492 ) ) ;
#66972=CARTESIAN_POINT ( 'NONE',  ( 34.56964662923419240, -285.9292752154952382, -293.5575057481635213 ) ) ;
#66973=CARTESIAN_POINT ( 'NONE',  ( 24.36765778347885103, -276.1647972375599238, -316.4149467717384141 ) ) ;
#66974=CARTESIAN_POINT ( 'NONE',  ( -82.74914644617162196, -293.4082697403888460, -211.0503515312420575 ) ) ;
#66976=CARTESIAN_POINT ( 'NONE',  ( -69.91165696735023971, -282.1233781216988064, -202.8022627189028810 ) ) ;
#66978=CARTESIAN_POINT ( 'NONE',  ( -106.9680502258036938, -276.1835217548601236, -298.6842498030480328 ) ) ;
#66980=CARTESIAN_POINT ( 'NONE',  ( -57.16178524344420708, -296.2006026990770238, -196.7292158022059141 ) ) ;
#66981=CARTESIAN_POINT ( 'NONE',  ( -97.92301971794994131, -272.4696893868625693, -229.3587696319173403 ) ) ;
#66982=AXIS2_PLACEMENT_3D ( 'NONE', #33791, #19122, #3037 ) ;
#66983=CARTESIAN_POINT ( 'NONE',  ( -108.7853764634695324, -292.3091231213562082, -252.2401853915949346 ) ) ;
#66984=CARTESIAN_POINT ( 'NONE',  ( -52.42991519985337590, -292.7955404200284306, -198.6448713283560892 ) ) ;
#66985=CARTESIAN_POINT ( 'NONE',  ( -99.87536134978427071, -285.7715062841502913, -310.0488776312305390 ) ) ;
#66986=CARTESIAN_POINT ( 'NONE',  ( -1.099458937905831046, -293.9488008365583482, -203.0922080215096912 ) ) ;
#66987=CARTESIAN_POINT ( 'NONE',  ( 10.79542237820755801, -294.0166852179127659, -210.8277229195600739 ) ) ;
#66988=CARTESIAN_POINT ( 'NONE',  ( 10.28991587961307808, -294.2063519485525944, -325.6804560207181680 ) ) ;
#66989=CARTESIAN_POINT ( 'NONE',  ( 4.757764759355538331, -290.4842402628768809, -332.4933580632563235 ) ) ;
#66990=CARTESIAN_POINT ( 'NONE',  ( 35.60976771557110965, -282.0310421820111628, -295.1658925406056824 ) ) ;
#66991=CARTESIAN_POINT ( 'NONE',  ( -101.6577801209563603, -271.2242178407157098, -230.3143037071844788 ) ) ;
#66992=CARTESIAN_POINT ( 'NONE',  ( -95.81516978679371732, -285.0621525138377024, -220.1827133802016192 ) ) ;
#66994=CARTESIAN_POINT ( 'NONE',  ( 17.76202262981522040, -278.2385657843595936, -320.7332088602555586 ) ) ;
#66995=CARTESIAN_POINT ( 'NONE',  ( -108.7482648970749182, -283.5704796478498224, -253.3296122133066319 ) ) ;
#66996=CARTESIAN_POINT ( 'NONE',  ( 34.03631996487620626, -285.8492817032945936, -293.3867319003311422 ) ) ;
#66997=CARTESIAN_POINT ( 'NONE',  ( -38.13285378101332412, -278.1819267755583382, -194.6004450691214629 ) ) ;
#66998=DIRECTION ( 'NONE',  ( 0.000000000000000000, 0.000000000000000000, 1.000000000000000000 ) ) ;
#66999=CARTESIAN_POINT ( 'NONE',  ( -104.6518066812248691, -284.4424024861571638, -241.8174135537645384 ) ) ;
#67001=CARTESIAN_POINT ( 'NONE',  ( -50.88458104402136684, -281.0878689522181162, -194.9648376097752305 ) ) ;
#67002=CARTESIAN_POINT ( 'NONE',  ( 38.44072848535298448, -286.7685144958991827, -282.9250486333608592 ) ) ;
#67003=CARTESIAN_POINT ( 'NONE',  ( 17.85098030138730607, -296.0081874964122903, -319.6929294394686849 ) ) ;
#67004=CARTESIAN_POINT ( 'NONE',  ( -9.485102557075622443, -278.2942285080972624, -341.2867860252569017 ) ) ;
#67005=CARTESIAN_POINT ( 'NONE',  ( 21.36306452885605012, -277.5317845536938535, -319.4228024309114176 ) ) ;
#67006=CARTESIAN_POINT ( 'NONE',  ( -40.50789072475588171, -276.9263566499165563, -343.3048872462796339 ) ) ;
#67007=CARTESIAN_POINT ( 'NONE',  ( 10.36552654395365991, -300.6508398382715086, -195.5114658272372026 ) ) ;
#67008=CARTESIAN_POINT ( 'NONE',  ( 31.66192681710618828, -285.1714003743475701, -241.2694682481871382 ) ) ;
#67009=CARTESIAN_POINT ( 'NONE',  ( -111.2239763421976591, -292.3886879039816904, -251.6577748456057009 ) ) ;
#67011=CARTESIAN_POINT ( 'NONE',  ( 6.235694213800440977, -293.3654088854264046, -329.3755113720337135 ) ) ;
#67013=CARTESIAN_POINT ( 'NONE',  ( 27.17476342466528294, -293.6859328467060095, -304.6702287837336485 ) ) ;
#67014=CARTESIAN_POINT ( 'NONE',  ( -69.50611118704075864, -292.7183612831727828, -200.7268419830291180 ) ) ;
#67015=CARTESIAN_POINT ( 'NONE',  ( -110.0043858952703602, -279.0922718530686097, -278.8098239488264767 ) ) ;
#67016=CARTESIAN_POINT ( 'NONE',  ( -102.5129343499546479, -272.1432336441174016, -229.7959797157119510 ) ) ;
#67017=CARTESIAN_POINT ( 'NONE',  ( 39.50290023730125455, -288.2542591529239075, -274.4092868848603644 ) ) ;
#67018=CARTESIAN_POINT ( 'NONE',  ( 0.7125367929813983814, -288.8927725998009919, -337.3363715993124856 ) ) ;
#67019=CARTESIAN_POINT ( 'NONE',  ( -68.78788600754154459, -285.9602766895080208, -204.4441763113638899 ) ) ;
#67020=CARTESIAN_POINT ( 'NONE',  ( 121.2562179577859354, 149.7689830918628218, -263.4557525057824137 ) ) ;
#67021=CARTESIAN_POINT ( 'NONE',  ( -23.55173957530102413, -107.6722516029799976, -361.1105106771343571 ) ) ;
#67022=CARTESIAN_POINT ( 'NONE',  ( -111.3618521999193689, -270.7884898157561793, -270.3386623361540160 ) ) ;
#67023=CARTESIAN_POINT ( 'NONE',  ( -39.17202761408243106, -276.2728720065729249, -343.4996962346045279 ) ) ;
#67024=CARTESIAN_POINT ( 'NONE',  ( -76.53263985705950745, -276.5099263182078744, -332.3748119067287803 ) ) ;
#67025=CARTESIAN_POINT ( 'NONE',  ( -23.36741030153408616, -297.7303750467191321, -193.4237862816653148 ) ) ;
#67026=CARTESIAN_POINT ( 'NONE',  ( 162.2625608158381851, 217.6175415146854561, -203.0404916468470446 ) ) ;
#67027=CARTESIAN_POINT ( 'NONE',  ( -95.78339516023345368, -276.5673149934908110, -319.7561003446909922 ) ) ;
#67028=CARTESIAN_POINT ( 'NONE',  ( 18.79638618443841125, -296.0184493717335386, -321.6480315517689519 ) ) ;
#67030=CARTESIAN_POINT ( 'NONE',  ( -100.3538522217745879, -290.5359661716732376, -307.4398937053138070 ) ) ;
#67031=CARTESIAN_POINT ( 'NONE',  ( -105.1160131458998990, -297.8251019792894567, -234.0432288662204314 ) ) ;
#67032=CARTESIAN_POINT ( 'NONE',  ( -63.53018616911869287, -274.3710191716231179, -198.0598317881868695 ) ) ;
#67033=CARTESIAN_POINT ( 'NONE',  ( -110.2415590959016782, -296.6684097743927850, -274.1834951170034742 ) ) ;
#67037=CARTESIAN_POINT ( 'NONE',  ( -100.8727300690507747, -279.9242658994360795, -311.3603658274947179 ) ) ;
#67038=CARTESIAN_POINT ( 'NONE',  ( 26.66720809742409770, -281.6221709145204954, -313.0505378778299246 ) ) ;
#67040=CARTESIAN_POINT ( 'NONE',  ( -110.4756489247802307, -279.5562228984588842, -276.1167851085758116 ) ) ;
#67041=CARTESIAN_POINT ( 'NONE',  ( -113.2189234111708629, -280.2606260639273614, -274.4380038564601705 ) ) ;
#67042=CARTESIAN_POINT ( 'NONE',  ( -102.6358645727413546, -271.4939527721521699, -236.0837082406988827 ) ) ;
#67045=CARTESIAN_POINT ( 'NONE',  ( 25.13518729998423495, -281.1979333874322720, -232.5055345102541082 ) ) ;
#67047=CARTESIAN_POINT ( 'NONE',  ( 34.03805652046323615, -276.7182139850921772, -298.9491097672543560 ) ) ;
#67048=CARTESIAN_POINT ( 'NONE',  ( 30.72691149552677459, -277.1372324023639635, -238.7468250872570934 ) ) ;
#67049=CARTESIAN_POINT ( 'NONE',  ( 38.14833764748937028, -273.9767750546992033, -258.4503894650110283 ) ) ;
#67052=CARTESIAN_POINT ( 'NONE',  ( 28.34087215466204768, -284.0229137394446752, -307.4026926134327482 ) ) ;
#67053=CIRCLE ( 'NONE', #26226, 2.500000000000002220 ) ;
#67054=CARTESIAN_POINT ( 'NONE',  ( -64.12121758476423850, -290.8908356855160946, -202.2633493847105512 ) ) ;
#67055=CARTESIAN_POINT ( 'NONE',  ( 9.754876809975540297, -286.0300808005186468, -209.5727537424507148 ) ) ;
#67056=EDGE_CURVE ( 'NONE', #52349, #64758, #86952, .T. ) ;
#67057=CARTESIAN_POINT ( 'NONE',  ( -38.92897890924263038, -281.3121561975418672, -344.3700964878531181 ) ) ;
#67058=CARTESIAN_POINT ( 'NONE',  ( -48.43527695111280451, -281.7708530120160617, -343.1093651726184817 ) ) ;
#67059=CARTESIAN_POINT ( 'NONE',  ( 3.252362589439977469, -284.6821418321059127, -207.9637120391448946 ) ) ;
#67060=CARTESIAN_POINT ( 'NONE',  ( -16.82534786963879014, -281.5282079434873594, -199.8897777521180217 ) ) ;
#67061=CARTESIAN_POINT ( 'NONE',  ( -31.84918176365186682, -124.6684167596312136, -365.2437734796851601 ) ) ;
#67062=CARTESIAN_POINT ( 'NONE',  ( -78.74234220796599004, -281.9998775941510303, -334.3331997810662983 ) ) ;
#67063=CARTESIAN_POINT ( 'NONE',  ( -4.091918615892772060, -296.6139714275789743, -337.6022192395366233 ) ) ;
#67065=CARTESIAN_POINT ( 'NONE',  ( -38.13652149106722078, -278.2821852550586073, -194.3786050189345644 ) ) ;
#67066=CARTESIAN_POINT ( 'NONE',  ( -89.15221949020558156, -278.4558738240499451, -322.0039394398951913 ) ) ;
#67067=CARTESIAN_POINT ( 'NONE',  ( -79.92116755735197842, -287.4782616339509218, -208.3546154443345984 ) ) ;
#67069=CARTESIAN_POINT ( 'NONE',  ( -5.238584658564489516, -294.3914906410022923, -201.9600640479076787 ) ) ;
#67071=CARTESIAN_POINT ( 'NONE',  ( 37.00639414487677925, -273.4252965533545421, -260.4939235253460765 ) ) ;
#67072=CARTESIAN_POINT ( 'NONE',  ( 12.30369635928613192, -287.5782853685344094, -329.0083125243459108 ) ) ;
#67073=CARTESIAN_POINT ( 'NONE',  ( 15.46200124246062302, -291.2135156333661712, -218.7300750239710965 ) ) ;
#67074=DIRECTION ( 'NONE',  ( -1.000000000000000000, -0.000000000000000000, -0.000000000000000000 ) ) ;
#67075=CARTESIAN_POINT ( 'NONE',  ( -61.97076326710509875, -276.0638323838589372, -339.6586574966509602 ) ) ;
#67076=CARTESIAN_POINT ( 'NONE',  ( -101.2415784662805152, -294.1800223847569100, -308.2469228993342085 ) ) ;
#67077=CARTESIAN_POINT ( 'NONE',  ( -107.4172661429287814, -291.5736688567221222, -292.6801288580591631 ) ) ;
#67078=DIRECTION ( 'NONE',  ( -5.501794166262391869E-14, -0.01273136352371387336, 0.9999189529070978688 ) ) ;
#67080=CARTESIAN_POINT ( 'NONE',  ( -6.152451996253581967, -290.9344534533494198, -200.7054560148281439 ) ) ;
#67081=CARTESIAN_POINT ( 'NONE',  ( 0.5622441613669305616, -288.1661762795995969, -206.9791093043430976 ) ) ;
#67082=CARTESIAN_POINT ( 'NONE',  ( -111.0066043073602202, -289.0289617690413593, -251.6686016540460287 ) ) ;
#67084=CARTESIAN_POINT ( 'NONE',  ( -6.788291178628715450, -287.8865278912126087, -203.4005563017663292 ) ) ;
#67086=CARTESIAN_POINT ( 'NONE',  ( 35.15473015238328003, -288.2205742338979917, -260.1492372354751410 ) ) ;
#67087=CARTESIAN_POINT ( 'NONE',  ( -87.49159065223909693, -297.7272680495831878, -326.6751383333937611 ) ) ;
#67089=CARTESIAN_POINT ( 'NONE',  ( 34.70428713649813091, -289.0893596023928467, -296.5421444732897953 ) ) ;
#67090=CARTESIAN_POINT ( 'NONE',  ( -56.12183050692097908, -277.8316678855341024, -197.3298115186908603 ) ) ;
#67091=CARTESIAN_POINT ( 'NONE',  ( -99.63015502882376495, -278.2848947340166319, -315.6150755841263162 ) ) ;
#67092=CARTESIAN_POINT ( 'NONE',  ( 24.57726242904086078, -280.6108963186658798, -224.6250669129683786 ) ) ;
#67093=CARTESIAN_POINT ( 'NONE',  ( -101.3192648241746809, -299.0506401058523807, -231.8064421044385881 ) ) ;
#67094=CARTESIAN_POINT ( 'NONE',  ( -11.30440954584355140, -284.3912514542718100, -200.0257773101257328 ) ) ;
#67096=CARTESIAN_POINT ( 'NONE',  ( -69.02940375500685377, -277.7704813289437311, -203.2287493168912249 ) ) ;
#67097=CARTESIAN_POINT ( 'NONE',  ( -96.48345021416767509, -281.9193463663916077, -316.4832823921498743 ) ) ;
#67099=CARTESIAN_POINT ( 'NONE',  ( 33.53302209126650268, -274.3956334448254211, -298.7785890836640306 ) ) ;
#67100=CARTESIAN_POINT ( 'NONE',  ( -58.58982259336092824, -296.8520811827672219, -340.9247420584073893 ) ) ;
#67101=CARTESIAN_POINT ( 'NONE',  ( 0.7030212800304437293, -281.4775768392740360, -336.9652633126052592 ) ) ;
#67102=CARTESIAN_POINT ( 'NONE',  ( -66.92534439354429310, -298.5959352864591096, -203.3532405654270860 ) ) ;
#67103=CARTESIAN_POINT ( 'NONE',  ( -66.02301925929761239, -275.1093884928051807, -199.5234128694778235 ) ) ;
#67104=CARTESIAN_POINT ( 'NONE',  ( -90.20898637332717840, -272.9452320430669943, -219.9728193391177342 ) ) ;
#67105=CARTESIAN_POINT ( 'NONE',  ( 33.68713843373978989, -295.2389984390615041, -246.1184032491807443 ) ) ;
#67106=CARTESIAN_POINT ( 'NONE',  ( 38.55650100448199424, -287.5555370908015789, -257.3042308033624295 ) ) ;
#67107=CARTESIAN_POINT ( 'NONE',  ( -73.06288539889933986, -277.6624097925532624, -203.7633346351316845 ) ) ;
#67108=CARTESIAN_POINT ( 'NONE',  ( -91.60003651476441178, -289.6322510181590815, -325.0715803121302088 ) ) ;
#67109=CARTESIAN_POINT ( 'NONE',  ( -86.89738658733573118, -288.8205650247093672, -324.3524838485369060 ) ) ;
#67110=CARTESIAN_POINT ( 'NONE',  ( -25.31635262876623216, -290.2052931954627866, -196.3314505255221434 ) ) ;
#67114=CARTESIAN_POINT ( 'NONE',  ( -92.46227780242949734, -289.3759609834672801, -318.3920261567783427 ) ) ;
#67116=CARTESIAN_POINT ( 'NONE',  ( -43.65889435197683355, -286.9155621666130855, -193.8036862660932229 ) ) ;
#67117=CARTESIAN_POINT ( 'NONE',  ( 17.36665895637874613, -289.4090924074130839, -226.6919474004047572 ) ) ;
#67118=CARTESIAN_POINT ( 'NONE',  ( 37.22856853686766243, -292.8401845483138572, -288.6395646410342692 ) ) ;
#67119=CARTESIAN_POINT ( 'NONE',  ( 27.89332935335748687, -283.3940585929251483, -310.4326541464980664 ) ) ;
#67120=CARTESIAN_POINT ( 'NONE',  ( -62.56088033759416334, -285.5480941702116411, -201.8017877787754344 ) ) ;
#67121=CARTESIAN_POINT ( 'NONE',  ( -96.93742279020844421, -273.3736483458357043, -221.5824675792455594 ) ) ;
#67122=CARTESIAN_POINT ( 'NONE',  ( 29.61037270951217693, -277.2730852330810762, -300.6705788711578862 ) ) ;
#67123=CARTESIAN_POINT ( 'NONE',  ( -2.854407636615578614, -290.5304793409114268, -204.1608652479899035 ) ) ;
#67124=CARTESIAN_POINT ( 'NONE',  ( 28.22283236386519434, -273.9017473753379477, -237.3698678889065548 ) ) ;
#67126=CARTESIAN_POINT ( 'NONE',  ( -90.78337343436103879, -230.3218577325732781, -348.1307343985224634 ) ) ;
#67127=CARTESIAN_POINT ( 'NONE',  ( 23.14770022548389505, -288.8765671158278678, -226.8882310111470986 ) ) ;
#67129=CARTESIAN_POINT ( 'NONE',  ( -111.2902972993403239, -297.3761934605768715, -290.6859177791066600 ) ) ;
#67131=CARTESIAN_POINT ( 'NONE',  ( -79.37466418584727990, -286.1195492096652515, -210.4899178405654254 ) ) ;
#67132=CARTESIAN_POINT ( 'NONE',  ( -112.1696816401933461, -277.8258537772218801, -253.2265506668895512 ) ) ;
#67133=CARTESIAN_POINT ( 'NONE',  ( 37.32098186564452647, -293.9729947841724993, -251.9546869176466544 ) ) ;
#67134=CARTESIAN_POINT ( 'NONE',  ( -5.274848766114055287, -284.6092408817195860, -201.7169446826105741 ) ) ;
#67135=CARTESIAN_POINT ( 'NONE',  ( -32.00973624925237715, -295.3199247476409823, -347.1683429578675373 ) ) ;
#67136=CARTESIAN_POINT ( 'NONE',  ( -62.81207961219386959, -292.0444990326904531, -201.9261323706388680 ) ) ;
#67137=DIRECTION ( 'NONE',  ( -1.000000000000000000, -0.000000000000000000, -0.000000000000000000 ) ) ;
#67139=CARTESIAN_POINT ( 'NONE',  ( -69.44094709309867142, -196.3684237510412345, -356.8806884016054823 ) ) ;
#67140=CARTESIAN_POINT ( 'NONE',  ( -111.0565450862888923, -286.3236734884974908, -250.4435723626106096 ) ) ;
#67141=CARTESIAN_POINT ( 'NONE',  ( -111.2586520408596868, -276.4809262143062369, -234.7283546768995564 ) ) ;
#67143=CARTESIAN_POINT ( 'NONE',  ( -108.3962118054631389, -283.2353629247668891, -288.4022500083157183 ) ) ;
#67144=CARTESIAN_POINT ( 'NONE',  ( -107.3981177076023101, -278.6282213137575354, -238.3291488797613056 ) ) ;
#67145=CARTESIAN_POINT ( 'NONE',  ( 30.99887550291407479, -283.9542864923766956, -300.9776946793386401 ) ) ;
#67146=CARTESIAN_POINT ( 'NONE',  ( 204.7386030247377562, 293.0225492072176507, -68.45606671877085603 ) ) ;
#67147=CARTESIAN_POINT ( 'NONE',  ( -55.57926598438943699, -281.8571562876591088, -344.5635268580948605 ) ) ;
#67148=CARTESIAN_POINT ( 'NONE',  ( -41.38742328547321847, -284.0210952733966678, -195.8132526376336955 ) ) ;
#67149=CARTESIAN_POINT ( 'NONE',  ( -21.63436553773008697, -276.1118636618704727, -196.2423948563264560 ) ) ;
#67150=TOROIDAL_SURFACE ( 'NONE', #89747, 5.654241149514405151, 0.5000000000000000000 ) ;
#67151=CARTESIAN_POINT ( 'NONE',  ( -107.5202228255254511, -297.3130572852704745, -250.0396172073275807 ) ) ;
#67152=CARTESIAN_POINT ( 'NONE',  ( 35.32300509861118343, -292.3854889307983171, -281.6954669123883832 ) ) ;
#67153=CARTESIAN_POINT ( 'NONE',  ( -104.7082862754642889, -279.6844843211132456, -233.2793723770433871 ) ) ;
#67154=CARTESIAN_POINT ( 'NONE',  ( -39.15776283274031044, -277.0755747228943733, -343.3385248716291471 ) ) ;
#67155=CARTESIAN_POINT ( 'NONE',  ( -34.78126636156569873, -299.0247202028718334, -193.5960124504560156 ) ) ;
#67156=CARTESIAN_POINT ( 'NONE',  ( -42.79795384507593070, -276.0398226069784187, -346.8576656513618559 ) ) ;
#67157=CARTESIAN_POINT ( 'NONE',  ( -100.1937721120643232, -247.9095777054778296, -334.1646650126361351 ) ) ;
#67158=CARTESIAN_POINT ( 'NONE',  ( 3.986236950277149305, -274.4957818316621001, -333.0085410706611810 ) ) ;
#67160=CARTESIAN_POINT ( 'NONE',  ( 29.07159097861759633, -295.4731154986054094, -308.2553614361412428 ) ) ;
#67162=CARTESIAN_POINT ( 'NONE',  ( -110.2140130185359368, -271.2396475792842807, -270.3444066551136871 ) ) ;
#67163=CARTESIAN_POINT ( 'NONE',  ( -109.0194057203915179, -285.4290162551033063, -285.8003045221917660 ) ) ;
#67164=CARTESIAN_POINT ( 'NONE',  ( -93.63319914156471668, -285.6094369579729459, -321.4219724254002131 ) ) ;
#67165=CARTESIAN_POINT ( 'NONE',  ( -9.446826437434063806, -285.7751645927073696, -202.7771184128829134 ) ) ;
#67166=CARTESIAN_POINT ( 'NONE',  ( -94.54787670534862798, -277.6048834966633763, -223.7360841601449977 ) ) ;
#67167=CARTESIAN_POINT ( 'NONE',  ( -81.33948134609407532, -285.5175458894618714, -330.2168709138405234 ) ) ;
#67168=CARTESIAN_POINT ( 'NONE',  ( -71.24356140075919086, -278.0760311576885329, -204.9147077670567967 ) ) ;
#67169=CARTESIAN_POINT ( 'NONE',  ( -43.21821857092100316, -278.2077764581086399, -343.4343183007009088 ) ) ;
#67171=CARTESIAN_POINT ( 'NONE',  ( -87.38001200859233109, -273.8240679204694175, -217.0550541341134760 ) ) ;
#67172=CARTESIAN_POINT ( 'NONE',  ( 12.87889640766004362, -281.5354978606392820, -212.2057183741234496 ) ) ;
#67173=CARTESIAN_POINT ( 'NONE',  ( -2.423677066864237339, -280.9939176628369637, -201.7879707990360032 ) ) ;
#67177=CARTESIAN_POINT ( 'NONE',  ( 38.34233430548384547, -289.3554556185041520, -265.8676532450549530 ) ) ;
#67178=CARTESIAN_POINT ( 'NONE',  ( -57.94047622556596622, -296.9763115912165290, -200.1593220665804438 ) ) ;
#67179=CARTESIAN_POINT ( 'NONE',  ( -81.86460726792671494, -290.8115074242801370, -207.6632430096129269 ) ) ;
#67181=CARTESIAN_POINT ( 'NONE',  ( 30.60851312404269109, -285.6513616178258417, -241.7073793894672349 ) ) ;
#67182=CARTESIAN_POINT ( 'NONE',  ( -0.7137964244690365723, -287.1305112318431725, -334.2458695315031036 ) ) ;
#67183=CARTESIAN_POINT ( 'NONE',  ( -19.73538753594966266, -287.4886996175510490, -199.1070075008561560 ) ) ;
#67184=CARTESIAN_POINT ( 'NONE',  ( -87.88362010494839183, -275.7586119608566264, -325.7733456167005670 ) ) ;
#67185=CARTESIAN_POINT ( 'NONE',  ( -62.51875825914677876, -287.7741057323520408, -342.3374072339535701 ) ) ;
#67187=CARTESIAN_POINT ( 'NONE',  ( -66.43731475674965736, -287.6713123412391724, -201.2348143065191834 ) ) ;
#67188=CARTESIAN_POINT ( 'NONE',  ( -26.43631521522038597, -286.9135113304699303, -344.7324901920360389 ) ) ;
#67189=CARTESIAN_POINT ( 'NONE',  ( 27.06766247056771135, -282.9674346090739050, -305.2157081696362297 ) ) ;
#67190=CARTESIAN_POINT ( 'NONE',  ( -112.3597751268069374, -292.6128376636565349, -265.6370469035957740 ) ) ;
#67193=CARTESIAN_POINT ( 'NONE',  ( -37.62722966810062530, -299.9687512229966160, -194.8016534822850190 ) ) ;
#67194=CARTESIAN_POINT ( 'NONE',  ( 18.96691926186968402, -280.0881349738864969, -223.6304183291449590 ) ) ;
#67195=CARTESIAN_POINT ( 'NONE',  ( 31.13025227645281845, -279.9546092520665752, -301.0923321726776862 ) ) ;
#67196=CARTESIAN_POINT ( 'NONE',  ( 21.23790151372838864, -293.4210296920037422, -320.0862534018947372 ) ) ;
#67197=CARTESIAN_POINT ( 'NONE',  ( -69.58890371489638937, -296.0202478865766125, -203.9792056979342760 ) ) ;
#67198=CARTESIAN_POINT ( 'NONE',  ( 26.60023806229068555, -274.1459053420546752, -308.4759803933796434 ) ) ;
#67199=CARTESIAN_POINT ( 'NONE',  ( -7.774641969351842263, -295.9715550941667743, -337.6580151683760960 ) ) ;
#67201=CARTESIAN_POINT ( 'NONE',  ( -89.74545365340810577, -271.9052102155274042, -214.6790523281290177 ) ) ;
#67203=CARTESIAN_POINT ( 'NONE',  ( -66.55584663536464518, -293.6693983638438112, -340.5214651889994002 ) ) ;
#67204=CIRCLE ( 'NONE', #85376, 2.888540232138026020 ) ;
#67206=CARTESIAN_POINT ( 'NONE',  ( -32.13355566123360063, -293.5443747821661873, -196.9436946687442287 ) ) ;
#67208=CARTESIAN_POINT ( 'NONE',  ( 6.765473385440317067, -293.4727160591680786, -211.9902436436635185 ) ) ;
#67210=CARTESIAN_POINT ( 'NONE',  ( -111.9740461264605216, -282.4344743007750367, -281.1430340061093602 ) ) ;
#67211=CARTESIAN_POINT ( 'NONE',  ( 24.42725678660558941, -294.0907046220681877, -309.3610324079171505 ) ) ;
#67213=CARTESIAN_POINT ( 'NONE',  ( -61.23167197043027699, -283.3538578861689530, -343.6170021527532867 ) ) ;
#67214=CARTESIAN_POINT ( 'NONE',  ( 23.41894926102405705, -282.8639673083965249, -225.4449996485074053 ) ) ;
#67215=CARTESIAN_POINT ( 'NONE',  ( -20.98432085465331554, -285.9232626858099593, -195.1402403305374946 ) ) ;
#67216=CARTESIAN_POINT ( 'NONE',  ( -101.8980960154815563, -288.0438598959605656, -308.3116207361771330 ) ) ;
#67217=CARTESIAN_POINT ( 'NONE',  ( -112.3417001280813707, -270.0523547857346784, -270.3292895737545223 ) ) ;
#67218=CARTESIAN_POINT ( 'NONE',  ( 11.03793403273828133, -280.8766763805475648, -329.4389598514219983 ) ) ;
#67220=CARTESIAN_POINT ( 'NONE',  ( -81.76343465556995227, -284.1173616825222439, -211.8123948694205012 ) ) ;
#67221=CARTESIAN_POINT ( 'NONE',  ( -109.5790508519872759, -289.1443324696557511, -296.2724259491490102 ) ) ;
#67223=CARTESIAN_POINT ( 'NONE',  ( -87.01354922164073002, -297.3578301508761683, -324.9426883259619672 ) ) ;
#67224=CARTESIAN_POINT ( 'NONE',  ( -111.9054128004683548, -279.7669623011300928, -287.0601912528625235 ) ) ;
#67225=CARTESIAN_POINT ( 'NONE',  ( 30.73307997374178413, -291.9968334733025017, -302.7972363169708387 ) ) ;
#67226=CARTESIAN_POINT ( 'NONE',  ( -105.5325100142869701, -278.5692543396213523, -244.1024537456504788 ) ) ;
#67227=CARTESIAN_POINT ( 'NONE',  ( -36.27231987935523705, -295.2058083195963718, -347.3667955588527434 ) ) ;
#67228=CARTESIAN_POINT ( 'NONE',  ( -112.3865618798553214, -282.7442553626093513, -261.5530011744070293 ) ) ;
#67230=CARTESIAN_POINT ( 'NONE',  ( -73.11975142816839934, -279.5265209563599456, -336.2918238646853411 ) ) ;
#67231=CARTESIAN_POINT ( 'NONE',  ( -72.24724726191968216, -294.5846537082790633, -334.7571956517979288 ) ) ;
#67232=CARTESIAN_POINT ( 'NONE',  ( -36.19614810475733435, -296.0663354996369776, -195.3614998211027682 ) ) ;
#67235=CARTESIAN_POINT ( 'NONE',  ( 28.31347594401546530, -284.0059076043989421, -305.8751244430252996 ) ) ;
#67236=CARTESIAN_POINT ( 'NONE',  ( -73.33817941723678757, -295.0511172822161257, -333.9397458422032514 ) ) ;
#67238=CARTESIAN_POINT ( 'NONE',  ( -95.95921662488163406, -276.6952119285918457, -223.5744983911110353 ) ) ;
#67239=CARTESIAN_POINT ( 'NONE',  ( -0.1147036217591330398, -273.7315856037491812, -203.1277831806561949 ) ) ;
#67240=CARTESIAN_POINT ( 'NONE',  ( 38.60317270302880388, -288.9892022401427312, -280.0440473583533390 ) ) ;
#67241=CARTESIAN_POINT ( 'NONE',  ( -109.1792958072182671, -290.2143049699486710, -283.3364735291740431 ) ) ;
#67242=CARTESIAN_POINT ( 'NONE',  ( -96.97807113952106306, -280.6724213909766945, -227.0689592676622794 ) ) ;
#67243=CARTESIAN_POINT ( 'NONE',  ( -79.32675617718699357, -275.0753945812171537, -209.6055766035934198 ) ) ;
#67244=CARTESIAN_POINT ( 'NONE',  ( -83.67658917716417477, -278.1951032996797721, -213.3725173046678378 ) ) ;
#67246=CARTESIAN_POINT ( 'NONE',  ( -5.112330907720179063, -274.2981139810358400, -200.4306685046049950 ) ) ;
#67247=CARTESIAN_POINT ( 'NONE',  ( -2.993122102728259737, -294.4298949750158272, -204.3195448023802498 ) ) ;
#67248=FACE_OUTER_BOUND ( 'NONE', #76556, .T. ) ;
#67250=CARTESIAN_POINT ( 'NONE',  ( -11.55107514696371851, -290.5239656839238478, -199.0658906205357255 ) ) ;
#67251=CARTESIAN_POINT ( 'NONE',  ( -102.0820708704232374, -272.5215621517092472, -236.3890010556425807 ) ) ;
#67253=CARTESIAN_POINT ( 'NONE',  ( -112.6724754502308912, -291.9187502847668156, -282.5259049713156969 ) ) ;
#67254=CARTESIAN_POINT ( 'NONE',  ( -99.90806341382572953, -293.6948066931273047, -220.5068182859052968 ) ) ;
#67255=CARTESIAN_POINT ( 'NONE',  ( -42.83346622741892418, -287.9828744991214080, -195.7166207263345541 ) ) ;
#67256=CARTESIAN_POINT ( 'NONE',  ( 36.43735435630544117, -273.3899329068153747, -257.7676863724011014 ) ) ;
#67257=CARTESIAN_POINT ( 'NONE',  ( 34.64078572484808660, -277.7179406150380032, -289.3304598472988687 ) ) ;
#67258=CARTESIAN_POINT ( 'NONE',  ( 13.91200012302444478, -290.8578076680587401, -216.3761903949640555 ) ) ;
#67259=CARTESIAN_POINT ( 'NONE',  ( -2.971988806569705321, -282.3617651154215764, -202.8260506594240553 ) ) ;
#67261=CARTESIAN_POINT ( 'NONE',  ( 32.32593649537962222, -281.1958750550029436, -292.6689329687255281 ) ) ;
#67262=CARTESIAN_POINT ( 'NONE',  ( -111.1393078996293156, -279.3692440797518088, -291.2274927854888347 ) ) ;
#67263=CARTESIAN_POINT ( 'NONE',  ( 25.59529122134308565, -280.9272285817746706, -314.0527493271473531 ) ) ;
#67265=CARTESIAN_POINT ( 'NONE',  ( -39.94293719427697908, -278.0253002991465223, -347.0947659806677166 ) ) ;
#67267=CARTESIAN_POINT ( 'NONE',  ( 31.24071122881919393, -277.5070611841730397, -303.9353912762309164 ) ) ;
#67268=CARTESIAN_POINT ( 'NONE',  ( -109.1418805571601069, -287.0519495502701943, -270.3937649182068412 ) ) ;
#67269=ORIENTED_EDGE ( 'NONE', *, *, #79023, .F. ) ;
#67271=CARTESIAN_POINT ( 'NONE',  ( -112.0447869666070488, -298.6451428507188552, -263.1315240048948567 ) ) ;
#67272=CARTESIAN_POINT ( 'NONE',  ( -105.3948903130178962, -291.2669158378200791, -297.7551264675065568 ) ) ;
#67273=CARTESIAN_POINT ( 'NONE',  ( -10.68979705083230058, -274.7229177476033897, -340.0857396393666932 ) ) ;
#67274=CARTESIAN_POINT ( 'NONE',  ( -94.67874910501100771, -291.6292510843045420, -320.2253018222972401 ) ) ;
#67275=CARTESIAN_POINT ( 'NONE',  ( -79.58285403195604601, -290.8133633878157980, -210.6368811586985146 ) ) ;
#67276=CARTESIAN_POINT ( 'NONE',  ( 37.66104898046413751, -286.8444951715351863, -253.1528583090604911 ) ) ;
#67278=CARTESIAN_POINT ( 'NONE',  ( -109.5065926550581707, -282.7496501993414313, -285.8701209447646647 ) ) ;
#67279=CARTESIAN_POINT ( 'NONE',  ( -108.1227528478971323, -292.1188228251868964, -292.9119394171157182 ) ) ;
#67280=CARTESIAN_POINT ( 'NONE',  ( -98.67347127916190175, -283.5938607794312247, -229.5062333300321029 ) ) ;
#67281=CARTESIAN_POINT ( 'NONE',  ( 2.960517666304172124, -281.9204804679612266, -208.8429654764919690 ) ) ;
#67282=CARTESIAN_POINT ( 'NONE',  ( 38.32289856104132042, -288.3299839405026432, -257.3343895402467751 ) ) ;
#67283=CARTESIAN_POINT ( 'NONE',  ( -93.14125524420126112, -279.7143763054685905, -223.1783463849918689 ) ) ;
#67284=CARTESIAN_POINT ( 'NONE',  ( -4.759029756074045103, -291.2667666911273159, -201.0330694611046169 ) ) ;
#67286=CARTESIAN_POINT ( 'NONE',  ( -35.16308127904952840, -286.8816498190725497, -193.5403693128261295 ) ) ;
#67287=CARTESIAN_POINT ( 'NONE',  ( -89.84883142852483218, -285.8272468408390523, -214.0522923289053097 ) ) ;
#67288=CARTESIAN_POINT ( 'NONE',  ( -99.02989991117676993, -284.1783019344570107, -309.4886300914752155 ) ) ;
#67291=CARTESIAN_POINT ( 'NONE',  ( 35.88259758053153803, -295.1644425481560461, -250.8558501298463455 ) ) ;
#67292=CARTESIAN_POINT ( 'NONE',  ( -13.94885471067347282, -293.4396545293069494, -343.2039148475573711 ) ) ;
#67293=CARTESIAN_POINT ( 'NONE',  ( -72.96691608450511524, -276.5952928440348728, -334.3618929345729498 ) ) ;
#67294=CARTESIAN_POINT ( 'NONE',  ( -108.7908082757884358, -296.2634908557384392, -241.7867818651185985 ) ) ;
#67296=CARTESIAN_POINT ( 'NONE',  ( 35.52053631844697890, -292.1805740573273624, -281.7288762314842074 ) ) ;
#67297=CARTESIAN_POINT ( 'NONE',  ( -111.3875495933986173, -294.8137731126849985, -268.6879279365750790 ) ) ;
#67298=CARTESIAN_POINT ( 'NONE',  ( -9.591502407463080360, -293.6279427758239535, -202.3581166651847809 ) ) ;
#67299=CARTESIAN_POINT ( 'NONE',  ( 33.94513861798802168, -294.4065384265440457, -253.2074537107375534 ) ) ;
#67301=CARTESIAN_POINT ( 'NONE',  ( -36.32541098104073996, -293.0393184409966238, -345.5337104244158013 ) ) ;
#67302=CARTESIAN_POINT ( 'NONE',  ( -96.11546781232344472, -299.1925850660058472, -223.7507064996990778 ) ) ;
#67303=CARTESIAN_POINT ( 'NONE',  ( -5.679891024229594798, -289.5664534029010611, -336.3985186978775346 ) ) ;
#67304=CARTESIAN_POINT ( 'NONE',  ( -56.48138831106356150, -279.2773817837849037, -343.2990007930033016 ) ) ;
#67305=CARTESIAN_POINT ( 'NONE',  ( 0.8357529046719096577, -275.3499996425079530, -336.8328046694530826 ) ) ;
#67306=CARTESIAN_POINT ( 'NONE',  ( -83.51225683111574938, -272.7865010018898033, -208.7998246219504779 ) ) ;
#67307=CARTESIAN_POINT ( 'NONE',  ( 6.419271446187398311, -280.5322395701727487, -330.5798157605046299 ) ) ;
#67308=CARTESIAN_POINT ( 'NONE',  ( -37.14965647360055812, -275.4496292092017029, -346.5738013586403099 ) ) ;
#67309=CARTESIAN_POINT ( 'NONE',  ( -105.2112596496005636, -295.6125463628455350, -242.1659700456739017 ) ) ;
#67310=CARTESIAN_POINT ( 'NONE',  ( -50.04721132641633830, -275.8903207208568915, -196.3932448144565512 ) ) ;
#67311=CARTESIAN_POINT ( 'NONE',  ( -74.33211428911454277, -274.1980928052942090, -207.2501019291577791 ) ) ;
#67312=DIRECTION ( 'NONE',  ( 0.000000000000000000, 1.000000000000000000, 8.326672684688666165E-15 ) ) ;
#67313=CARTESIAN_POINT ( 'NONE',  ( -112.6096505921947539, -288.5259291955848084, -273.9863673556396861 ) ) ;
#67314=CARTESIAN_POINT ( 'NONE',  ( -19.26957063406313964, -274.1244116509696482, -199.5810569675059014 ) ) ;
#67315=CARTESIAN_POINT ( 'NONE',  ( 37.50441561134613266, -287.7789892848617228, -288.5015900819303738 ) ) ;
#67316=CARTESIAN_POINT ( 'NONE',  ( -23.75605052931431516, -300.2013042008109096, -195.0013520409553109 ) ) ;
#67317=CARTESIAN_POINT ( 'NONE',  ( -97.56084291798067909, -295.1596666401516131, -225.9133383879100734 ) ) ;
#67318=CARTESIAN_POINT ( 'NONE',  ( -0.4619413555700691565, -281.7719555207291933, -337.7855361320704333 ) ) ;
#67320=CARTESIAN_POINT ( 'NONE',  ( 36.78398702179362800, -279.4043088283045790, -258.8592749498809553 ) ) ;
#67322=CARTESIAN_POINT ( 'NONE',  ( -94.59102870938559704, -289.9929276234884696, -224.4102804452266753 ) ) ;
#67323=CARTESIAN_POINT ( 'NONE',  ( -37.56767838799788706, -281.1946303143575960, -344.6086179463206349 ) ) ;
#67326=CARTESIAN_POINT ( 'NONE',  ( -112.2414146217796969, -288.6133317072296904, -265.5835082708381378 ) ) ;
#67327=CARTESIAN_POINT ( 'NONE',  ( -24.49441223519213295, -275.7390851462669161, -197.7442091394081274 ) ) ;
#67328=CARTESIAN_POINT ( 'NONE',  ( -61.09389884139567073, -284.5587395081295767, -343.2439904538098290 ) ) ;
#67329=CARTESIAN_POINT ( 'NONE',  ( 10.88574893284359923, -272.7926532337679078, -212.1258744927253588 ) ) ;
#67330=CARTESIAN_POINT ( 'NONE',  ( -107.3549595134004306, -284.8277144478067271, -249.5183499439539787 ) ) ;
#67331=CARTESIAN_POINT ( 'NONE',  ( 34.16335719649052294, -277.2056586243123775, -287.8039562352511780 ) ) ;
#67332=CARTESIAN_POINT ( 'NONE',  ( 29.30556371658614978, -276.7608262536016923, -300.5396525469514017 ) ) ;
#67334=CARTESIAN_POINT ( 'NONE',  ( -44.21001317057650226, -285.1390435861709420, -345.0979394246302832 ) ) ;
#67337=CARTESIAN_POINT ( 'NONE',  ( -114.3379425117592945, -296.3949860655756652, -269.6004187791383515 ) ) ;
#67338=CARTESIAN_POINT ( 'NONE',  ( 31.46843160601511968, -289.1508124478490913, -241.2961993220737611 ) ) ;
#67340=CARTESIAN_POINT ( 'NONE',  ( -99.86837403722181250, -294.6952119285919025, -220.4570493818173702 ) ) ;
#67341=CARTESIAN_POINT ( 'NONE',  ( -72.35338004339116935, -278.5202171850656327, -202.1140212282637094 ) ) ;
#67342=CARTESIAN_POINT ( 'NONE',  ( -99.36788428090561354, -289.5444752506206783, -226.0983469922730649 ) ) ;
#67343=CARTESIAN_POINT ( 'NONE',  ( -102.8636058403824762, -286.5264540420590720, -236.6329750986399461 ) ) ;
#67345=CARTESIAN_POINT ( 'NONE',  ( -72.63234576131131348, -281.3382144144436552, -205.3031104377008376 ) ) ;
#67346=CARTESIAN_POINT ( 'NONE',  ( -73.35150324320090931, -287.0097691400226836, -202.9088870676524436 ) ) ;
#67347=CARTESIAN_POINT ( 'NONE',  ( 27.29527643271218906, -284.0620442482561998, -308.5040672663332657 ) ) ;
#67348=CARTESIAN_POINT ( 'NONE',  ( 37.59235998408419022, -275.9410578058916599, -288.1347638980677175 ) ) ;
#67349=CARTESIAN_POINT ( 'NONE',  ( -47.47155398077692467, -295.9430146026742818, -196.3544935559752673 ) ) ;
#67350=CARTESIAN_POINT ( 'NONE',  ( -111.3366591557671370, -278.6525445484331271, -249.0598024596567370 ) ) ;
#67351=CARTESIAN_POINT ( 'NONE',  ( -71.14284257855211990, -299.5226429488563440, -204.0235030947206099 ) ) ;
#67354=CARTESIAN_POINT ( 'NONE',  ( -15.23521048091404140, -296.4656831749665571, -194.6032272679434243 ) ) ;
#67355=DIRECTION ( 'NONE',  ( 0.000000000000000000, 0.000000000000000000, 1.000000000000000000 ) ) ;
#67356=CARTESIAN_POINT ( 'NONE',  ( -80.86105611716482144, -277.1688461107187322, -329.0471818799301786 ) ) ;
#67357=CARTESIAN_POINT ( 'NONE',  ( -5.294431581063172132, -275.6696478140756312, -200.7839572271229542 ) ) ;
#67358=CARTESIAN_POINT ( 'NONE',  ( 32.17420931639730242, -281.0305581380645208, -303.0494582179358076 ) ) ;
#67359=CARTESIAN_POINT ( 'NONE',  ( 27.93461205222396160, -289.7825920756228015, -305.3554566858161934 ) ) ;
#67360=CARTESIAN_POINT ( 'NONE',  ( -66.64017007673201931, -296.9491317606980374, -340.8330313381994756 ) ) ;
#67361=CARTESIAN_POINT ( 'NONE',  ( -83.93147881670488175, -296.8808695817414218, -331.2342463426401196 ) ) ;
#67362=CARTESIAN_POINT ( 'NONE',  ( 36.28241170012432804, -295.3789794690508188, -256.8915399723416044 ) ) ;
#67363=CARTESIAN_POINT ( 'NONE',  ( 37.53694440331400273, -279.5648804297883885, -271.3631033876093284 ) ) ;
#67364=CARTESIAN_POINT ( 'NONE',  ( -30.14707827695709597, -282.0639053194449275, -196.2182614113812633 ) ) ;
#67365=CARTESIAN_POINT ( 'NONE',  ( -101.1181405841077918, -295.1512220851134316, -231.8697869987369700 ) ) ;
#67366=CARTESIAN_POINT ( 'NONE',  ( -105.0637131644742226, -285.6960084731403526, -305.4071083088259684 ) ) ;
#67367=CARTESIAN_POINT ( 'NONE',  ( -63.94584268494079993, -288.3276366471973233, -338.7269245778006166 ) ) ;
#67368=CARTESIAN_POINT ( 'NONE',  ( 123.3741230786721701, 148.3115526884368762, -263.0448026886833759 ) ) ;
#67370=CARTESIAN_POINT ( 'NONE',  ( 16.25958489967095488, -286.8843587642941770, -324.8911590190015772 ) ) ;
#67371=CARTESIAN_POINT ( 'NONE',  ( 35.01768728057285074, -287.0846437347926212, -260.1831399919752812 ) ) ;
#67373=CARTESIAN_POINT ( 'NONE',  ( -66.44615608580583910, -284.5041065694489930, -341.3289147227118292 ) ) ;
#67374=CARTESIAN_POINT ( 'NONE',  ( 26.65301224073414232, -275.4039328342498152, -235.0880852607534166 ) ) ;
#67375=CARTESIAN_POINT ( 'NONE',  ( -95.41779936946916507, -290.1517639958345853, -220.2545327573945144 ) ) ;
#67376=CARTESIAN_POINT ( 'NONE',  ( 26.64168061165032597, -282.7657468029810275, -313.0160095621785104 ) ) ;
#67377=CARTESIAN_POINT ( 'NONE',  ( -5.253321675605685748, -281.9869382675909151, -201.1293064831605193 ) ) ;
#67378=CARTESIAN_POINT ( 'NONE',  ( 39.39029413338710128, -281.8083722989147191, -264.2011384277763568 ) ) ;
#67379=CARTESIAN_POINT ( 'NONE',  ( 23.68253067946291779, -280.9956187450828793, -230.2069670555943333 ) ) ;
#67380=CARTESIAN_POINT ( 'NONE',  ( 10.59707575819633618, -273.9094976428776249, -330.5268031993606428 ) ) ;
#67381=CARTESIAN_POINT ( 'NONE',  ( 65.59659910285013495, 47.55397664594911333, -319.0097190562326546 ) ) ;
#67383=CARTESIAN_POINT ( 'NONE',  ( -13.16970484266629704, -278.7377274720011542, -341.2375088096205218 ) ) ;
#67384=CARTESIAN_POINT ( 'NONE',  ( -114.2697886859462244, -273.0835924068001077, -270.3678844897593194 ) ) ;
#67385=CARTESIAN_POINT ( 'NONE',  ( 36.99273977470537744, -279.4774700638589024, -263.0139704377475596 ) ) ;
#67386=CARTESIAN_POINT ( 'NONE',  ( -71.70559143042845562, -296.9340132534039753, -205.8254655126555974 ) ) ;
#67387=CARTESIAN_POINT ( 'NONE',  ( 38.54454576316462067, -293.2195243526579702, -283.1217813854034375 ) ) ;
#67388=CARTESIAN_POINT ( 'NONE',  ( 202.9739431815424950, 291.9636489454802017, -68.24819713444452418 ) ) ;
#67390=CARTESIAN_POINT ( 'NONE',  ( -59.95625032498254114, -296.3395747251707348, -197.3184347503279525 ) ) ;
#67391=CARTESIAN_POINT ( 'NONE',  ( -58.94253714722416504, -287.7360410946706111, -340.9825175202570904 ) ) ;
#67392=CARTESIAN_POINT ( 'NONE',  ( -103.8646930921256057, -297.9719881625472340, -303.4249985040450497 ) ) ;
#67394=CARTESIAN_POINT ( 'NONE',  ( -6.826924175246609217, -287.7764474206499585, -203.4885541252969006 ) ) ;
#67396=CARTESIAN_POINT ( 'NONE',  ( 38.99081327116950035, -294.3852573785742948, -261.7403986828321081 ) ) ;
#67397=CARTESIAN_POINT ( 'NONE',  ( -67.80431599386086816, -283.9554626635209047, -336.7690804303391019 ) ) ;
#67398=CARTESIAN_POINT ( 'NONE',  ( -31.92891780758167641, -296.9134330854134305, -193.7592673089102391 ) ) ;
#67399=CARTESIAN_POINT ( 'NONE',  ( -3.401908195211420072, -293.2916676576797954, -201.4100516542314949 ) ) ;
#67400=CARTESIAN_POINT ( 'NONE',  ( 15.39142019867240130, -293.2656090547933445, -214.2634698685775447 ) ) ;
#67401=CARTESIAN_POINT ( 'NONE',  ( -45.36034040768231534, -289.3232569012757835, -342.9193801762237968 ) ) ;
#67404=CARTESIAN_POINT ( 'NONE',  ( -75.18384841405867292, -299.4142964258866755, -204.6634285069642374 ) ) ;
#67405=CARTESIAN_POINT ( 'NONE',  ( -67.36580020186093520, -272.4619597697749782, -199.8872779138432918 ) ) ;
#67406=CARTESIAN_POINT ( 'NONE',  ( -36.20185349507786299, -282.0962594986025920, -343.5875421647188546 ) ) ;
#67408=CARTESIAN_POINT ( 'NONE',  ( -91.29036041939585289, -277.3019273465229162, -325.2907126768388366 ) ) ;
#67409=CARTESIAN_POINT ( 'NONE',  ( -64.84824277484651134, -272.0866938712898104, -201.8651549287907585 ) ) ;
#67410=CARTESIAN_POINT ( 'NONE',  ( -104.2339240973314105, -279.9828725069102120, -302.6715332450010010 ) ) ;
#67411=CARTESIAN_POINT ( 'NONE',  ( -41.95664951067705317, -275.2504754441462751, -344.4655445766188677 ) ) ;
#67412=CARTESIAN_POINT ( 'NONE',  ( -110.7718532313449344, -297.7785129490447957, -268.7393526505371142 ) ) ;
#67413=CARTESIAN_POINT ( 'NONE',  ( -54.27754474621303160, -274.7704907015208846, -199.1109557761341193 ) ) ;
#67414=CARTESIAN_POINT ( 'NONE',  ( -98.76140316746356973, -274.9149672771766859, -225.5346578042040733 ) ) ;
#67415=CARTESIAN_POINT ( 'NONE',  ( -10.90061306522138906, -272.4151549353603059, -199.7416152477110245 ) ) ;
#67416=CARTESIAN_POINT ( 'NONE',  ( 35.63586220609176536, -294.1369115335231754, -265.3010335679667833 ) ) ;
#67417=CARTESIAN_POINT ( 'NONE',  ( 15.30967845870372379, -291.3883435325480491, -218.8759821830510930 ) ) ;
#67419=CARTESIAN_POINT ( 'NONE',  ( 29.04601499248675367, -276.5510644160094103, -309.2481104629756601 ) ) ;
#67420=CARTESIAN_POINT ( 'NONE',  ( -67.05944909184545111, -273.8181155025218345, -203.6701768189681729 ) ) ;
#67422=CARTESIAN_POINT ( 'NONE',  ( -65.67903593495820758, -284.3740415478202976, -199.2816373236528591 ) ) ;
#67423=CARTESIAN_POINT ( 'NONE',  ( -1.556008960157877041, -296.5791324506783440, -336.4771845926472338 ) ) ;
#67425=CARTESIAN_POINT ( 'NONE',  ( -108.8204787368435120, -283.9554336488732815, -254.7018348278834026 ) ) ;
#67426=CARTESIAN_POINT ( 'NONE',  ( -102.8325016633909712, -282.0604138649675292, -307.3581083774112130 ) ) ;
#67427=CARTESIAN_POINT ( 'NONE',  ( 24.46952517151419926, -274.6764295799227966, -310.3893289985350066 ) ) ;
#67428=CARTESIAN_POINT ( 'NONE',  ( 35.95267868534529754, -283.7572755667330853, -286.3243486608157582 ) ) ;
#67432=CARTESIAN_POINT ( 'NONE',  ( 6.788450942039863989, -273.0409238516637060, -208.1757411893995311 ) ) ;
#67433=CARTESIAN_POINT ( 'NONE',  ( -111.9433666116181598, -280.4291977326778351, -279.9709956902827344 ) ) ;
#67435=CARTESIAN_POINT ( 'NONE',  ( -60.09994127140250697, -287.6797357710854044, -198.2553661509792278 ) ) ;
#67437=CARTESIAN_POINT ( 'NONE',  ( -97.00855831940396001, -289.1740740990533709, -224.8996233648030909 ) ) ;
#67439=CARTESIAN_POINT ( 'NONE',  ( -95.09533644216796233, -294.7118432871770324, -315.6562391179234055 ) ) ;
#67440=CARTESIAN_POINT ( 'NONE',  ( 12.97592401329083422, -286.4805591809691805, -325.0111833668403278 ) ) ;
#67441=CARTESIAN_POINT ( 'NONE',  ( -107.5886556134111913, -275.3214365662247474, -283.9876634089608274 ) ) ;
#67442=CARTESIAN_POINT ( 'NONE',  ( -35.04653889517396692, -296.0807262379776716, -195.3618917615749524 ) ) ;
#67443=CARTESIAN_POINT ( 'NONE',  ( 9.784413016715705069, -286.8969497366213659, -330.4436332668842056 ) ) ;
#67444=CARTESIAN_POINT ( 'NONE',  ( 19.11942211533632374, -283.8202233078185941, -317.9052839654305558 ) ) ;
#67445=CARTESIAN_POINT ( 'NONE',  ( -73.80962969314016675, -281.7689925138185458, -337.0836488720716488 ) ) ;
#67446=CARTESIAN_POINT ( 'NONE',  ( -37.54995011217922496, -292.0495095374964762, -197.3489713127045491 ) ) ;
#67447=CARTESIAN_POINT ( 'NONE',  ( 32.79842370658523265, -283.2722255939596607, -292.7923843633008687 ) ) ;
#67448=CARTESIAN_POINT ( 'NONE',  ( -3.537702344968634005, -283.3968537755233683, -335.2588312678752800 ) ) ;
#67449=CARTESIAN_POINT ( 'NONE',  ( -92.37396928192313794, -291.8139898961089216, -321.9130442082536661 ) ) ;
#67450=CARTESIAN_POINT ( 'NONE',  ( -68.17940801942711460, -297.8250554485802013, -199.7491228043520550 ) ) ;
#67451=CARTESIAN_POINT ( 'NONE',  ( -45.88765554208796260, -287.2394101657951069, -345.4884198094632097 ) ) ;
#67452=CARTESIAN_POINT ( 'NONE',  ( 21.85085722790037721, -274.8897807495739585, -221.1143804900233647 ) ) ;
#67453=CARTESIAN_POINT ( 'NONE',  ( -37.57995285703409394, -294.0290811345717543, -195.7039702635589151 ) ) ;
#67455=CARTESIAN_POINT ( 'NONE',  ( -110.4683760289727132, -287.2662352645559167, -253.7030783399848985 ) ) ;
#67456=CARTESIAN_POINT ( 'NONE',  ( -41.31366113791848704, -275.1018660200039676, -345.4356665749590434 ) ) ;
#67457=CARTESIAN_POINT ( 'NONE',  ( -111.4911300777384895, -295.1739438182590902, -252.8025742876987465 ) ) ;
#67458=CARTESIAN_POINT ( 'NONE',  ( -110.5809626054065404, -292.0338012384750641, -279.4413628334679629 ) ) ;
#67459=CARTESIAN_POINT ( 'NONE',  ( -48.88336149473123271, -273.2499681043040596, -198.1248148121722750 ) ) ;
#67460=CARTESIAN_POINT ( 'NONE',  ( -99.41545353577029687, -291.5280305657475424, -310.0795883700643003 ) ) ;
#67461=CARTESIAN_POINT ( 'NONE',  ( -83.98809387908922020, -292.3338723566047861, -213.9029706749503532 ) ) ;
#67462=CARTESIAN_POINT ( 'NONE',  ( -85.50444300002443754, -285.4891905527342146, -326.5600878139779866 ) ) ;
#67463=CARTESIAN_POINT ( 'NONE',  ( -74.40907086021208272, -292.9943638093243976, -203.5433335202371268 ) ) ;
#67464=CARTESIAN_POINT ( 'NONE',  ( -56.08429023104190492, -293.1309501595307552, -196.1309592579417256 ) ) ;
#67465=CARTESIAN_POINT ( 'NONE',  ( -38.34442247171282503, -294.8983877821257806, -343.3542310305479077 ) ) ;
#67466=CARTESIAN_POINT ( 'NONE',  ( 37.44837555031843834, -289.6327263595887302, -276.6236570827797436 ) ) ;
#67467=CARTESIAN_POINT ( 'NONE',  ( 37.33073559118222562, -281.4837439913778212, -251.5720959675283268 ) ) ;
#67468=CARTESIAN_POINT ( 'NONE',  ( -26.44372333233875949, -296.2674149621003608, -194.8046424488529738 ) ) ;
#67469=CARTESIAN_POINT ( 'NONE',  ( -64.54520477768802778, -285.5400060928985795, -198.3124494861497169 ) ) ;
#67470=CARTESIAN_POINT ( 'NONE',  ( 33.61770922075736934, -277.2294890997626453, -247.0301939133530595 ) ) ;
#67471=CARTESIAN_POINT ( 'NONE',  ( -109.8932374514378552, -283.1970374644556614, -281.7964063818723162 ) ) ;
#67472=CARTESIAN_POINT ( 'NONE',  ( 32.17862485025679575, -285.9204056158101253, -298.6404964028990321 ) ) ;
#67473=CARTESIAN_POINT ( 'NONE',  ( -68.52893239299793038, -275.5971571780453928, -339.4235526077253553 ) ) ;
#67475=CARTESIAN_POINT ( 'NONE',  ( -16.12061027350512887, -282.2778709951963378, -340.2728751261355455 ) ) ;
#67476=CARTESIAN_POINT ( 'NONE',  ( -6.404871329777954259, -281.6545982453667989, -200.2689547215233006 ) ) ;
#67477=CARTESIAN_POINT ( 'NONE',  ( 37.59263406070686386, -286.8206939588185946, -287.0843930966144626 ) ) ;
#67478=CARTESIAN_POINT ( 'NONE',  ( 18.75492264642632634, -295.9906309964503635, -318.6623604171315378 ) ) ;
#67479=CARTESIAN_POINT ( 'NONE',  ( 5.439153599253639726, -278.0835830056513487, -333.4185439391347927 ) ) ;
#67480=CARTESIAN_POINT ( 'NONE',  ( 25.67030322948781418, -277.4448831468405388, -313.8439183912683461 ) ) ;
#67481=CARTESIAN_POINT ( 'NONE',  ( -59.19702043671041736, -277.1763795744126924, -340.0127150833978931 ) ) ;
#67482=CARTESIAN_POINT ( 'NONE',  ( -99.99615301262304001, -299.1065787197618988, -229.3472803415267265 ) ) ;
#67483=CARTESIAN_POINT ( 'NONE',  ( 37.48819883521037610, -285.5612182979672298, -271.0785052673513746 ) ) ;
#67484=CARTESIAN_POINT ( 'NONE',  ( -98.37600032907307934, -291.5386813156269454, -316.0034578001072987 ) ) ;
#67485=CARTESIAN_POINT ( 'NONE',  ( 31.82715020783358284, -292.7960656610079013, -294.8008114295665223 ) ) ;
#67487=CARTESIAN_POINT ( 'NONE',  ( 19.36489469635971616, -292.5679730829990035, -224.3364538802302093 ) ) ;
#67489=CARTESIAN_POINT ( 'NONE',  ( -26.17592747168105660, -289.9928471740839768, -346.2348158631659203 ) ) ;
#67490=CARTESIAN_POINT ( 'NONE',  ( -32.96518863955563461, -280.7601599396897996, -197.3903100144099483 ) ) ;
#67491=CARTESIAN_POINT ( 'NONE',  ( -111.3202141966663135, -295.7289312489323834, -249.9493835531594925 ) ) ;
#67492=CARTESIAN_POINT ( 'NONE',  ( 20.20494462640257893, -287.5109782763636304, -219.2756966161275614 ) ) ;
#67493=CARTESIAN_POINT ( 'NONE',  ( -1.806709704085969870, -288.9276371305409725, -338.6473446111414773 ) ) ;
#67494=CARTESIAN_POINT ( 'NONE',  ( -65.31987339772369694, -283.7614687864306688, -337.8232879530835930 ) ) ;
#67495=CARTESIAN_POINT ( 'NONE',  ( -100.1937721120545604, -247.9095777054600660, -334.1646650126529039 ) ) ;
#67496=CARTESIAN_POINT ( 'NONE',  ( -110.6743395205602383, -264.9754415880684064, -306.3209493635451963 ) ) ;
#67497=CARTESIAN_POINT ( 'NONE',  ( 172.9423030596852300, 240.7948373491403800, -177.0476525864039274 ) ) ;
#67498=CARTESIAN_POINT ( 'NONE',  ( -72.92947600809826270, -276.7336899014498499, -334.2982353352063001 ) ) ;
#67499=CARTESIAN_POINT ( 'NONE',  ( -110.6598727148159185, -277.5050117346015668, -267.8841605835873452 ) ) ;
#67500=CARTESIAN_POINT ( 'NONE',  ( 76.28016853513979356, -298.9466307878727207, -193.4317762818265010 ) ) ;
#67501=CARTESIAN_POINT ( 'NONE',  ( -46.15978596236939779, -155.9775659802373582, -362.2499631079683695 ) ) ;
#67503=CARTESIAN_POINT ( 'NONE',  ( -28.67365081324876286, -275.6293807896831254, -346.4285795038637730 ) ) ;
#67505=CARTESIAN_POINT ( 'NONE',  ( -110.3075092998461884, -291.1054381300302225, -265.7379671348173247 ) ) ;
#67506=CARTESIAN_POINT ( 'NONE',  ( -57.35753066787983556, -298.6031769264931768, -196.1202044263708615 ) ) ;
#67507=CARTESIAN_POINT ( 'NONE',  ( 35.61173680904107641, -286.3534648892423888, -279.2515351168862594 ) ) ;
#67508=CARTESIAN_POINT ( 'NONE',  ( -33.34475477686601153, -298.5932824275707844, -193.4223321786282668 ) ) ;
#67509=CARTESIAN_POINT ( 'NONE',  ( -45.08862425399878049, -295.3195275842401202, -342.9993702803830047 ) ) ;
#67512=CARTESIAN_POINT ( 'NONE',  ( -41.28438838813088552, -279.0215473313475627, -345.8311498738309524 ) ) ;
#67513=CARTESIAN_POINT ( 'NONE',  ( 17.77780919329176612, -281.7970574513081488, -324.1155995742814184 ) ) ;
#67514=CARTESIAN_POINT ( 'NONE',  ( -85.29710753569284520, -278.8125153487922034, -325.8765691274239202 ) ) ;
#67515=CARTESIAN_POINT ( 'NONE',  ( -111.4906035245811893, -280.1017770074629425, -286.9717815096015556 ) ) ;
#67516=CARTESIAN_POINT ( 'NONE',  ( -101.3100796172653730, -271.5298930917532516, -233.6695579173734529 ) ) ;
#67518=CARTESIAN_POINT ( 'NONE',  ( -85.48577373792517164, -279.5307654605460357, -215.4871881001894849 ) ) ;
#67519=CARTESIAN_POINT ( 'NONE',  ( -102.5873322092470801, -273.8870371167427038, -229.7758212044883805 ) ) ;
#67520=CARTESIAN_POINT ( 'NONE',  ( -57.60636522454186803, -275.7908285814836518, -198.0967127139663546 ) ) ;
#67521=CARTESIAN_POINT ( 'NONE',  ( 7.877640444709827605, -275.0229685168492892, -332.0205893269721855 ) ) ;
#67523=CARTESIAN_POINT ( 'NONE',  ( -33.48973234059639026, -291.2990075363006213, -197.2885950236634756 ) ) ;
#67524=CARTESIAN_POINT ( 'NONE',  ( -111.6205801539287137, -284.1524892136673088, -250.2623046006208654 ) ) ;
#67525=CARTESIAN_POINT ( 'NONE',  ( 30.96519848262594721, -279.4149736307926446, -241.8630195639390763 ) ) ;
#67526=CARTESIAN_POINT ( 'NONE',  ( 7.515752311812053499, -279.2521724994480792, -211.9598184488929462 ) ) ;
#67527=CARTESIAN_POINT ( 'NONE',  ( -94.34228945494660934, -283.2987962867776446, -222.4837014149917991 ) ) ;
#67528=CARTESIAN_POINT ( 'NONE',  ( 28.10842582021338387, -290.0411469132703814, -307.0891890288916102 ) ) ;
#67529=CARTESIAN_POINT ( 'NONE',  ( 20.82122626363265994, -282.1303246469889814, -225.5723545549112714 ) ) ;
#67530=CARTESIAN_POINT ( 'NONE',  ( -80.08899952443231030, -271.4738533049682587, -208.6729679165025004 ) ) ;
#67531=CARTESIAN_POINT ( 'NONE',  ( 24.44652508566888471, -280.5498077183483474, -314.9776049113219187 ) ) ;
#67532=CARTESIAN_POINT ( 'NONE',  ( -19.73151157189154858, -296.8260355642370882, -343.3178187200014690 ) ) ;
#67533=CARTESIAN_POINT ( 'NONE',  ( -103.8951190663378981, -277.2733181421044151, -233.6921060075632397 ) ) ;
#67534=CARTESIAN_POINT ( 'NONE',  ( -71.69475909250618884, -278.1701329456275857, -334.9024402638229390 ) ) ;
#67535=CARTESIAN_POINT ( 'NONE',  ( -43.54108341269972726, -287.9742998348873471, -195.3985391084868297 ) ) ;
#67537=CARTESIAN_POINT ( 'NONE',  ( -47.57307327863838253, -293.8433565187115732, -195.4442292658428357 ) ) ;
#67538=CARTESIAN_POINT ( 'NONE',  ( 17.98991791078880453, -274.2591556012564524, -321.0104213023034845 ) ) ;
#67539=CARTESIAN_POINT ( 'NONE',  ( -74.35851822292511315, -288.7286195731140879, -337.7104857608807151 ) ) ;
#67540=CARTESIAN_POINT ( 'NONE',  ( 7.174846915916289092, -291.0701418209096687, -211.4992674139771509 ) ) ;
#67542=CARTESIAN_POINT ( 'NONE',  ( -3.656252300233240327, -275.2826617979363277, -335.6798295734435555 ) ) ;
#67543=CARTESIAN_POINT ( 'NONE',  ( -94.91529874919451970, -294.0392675413422126, -317.2441618246101598 ) ) ;
#67544=CARTESIAN_POINT ( 'NONE',  ( -99.24821154366281917, -291.3231156582584163, -309.9695428704239930 ) ) ;
#67547=CARTESIAN_POINT ( 'NONE',  ( 23.43485513168371170, -291.4113841519857715, -224.1994090858819675 ) ) ;
#67548=CARTESIAN_POINT ( 'NONE',  ( 31.23605002149735910, -289.5147929915862051, -297.7668382666107050 ) ) ;
#67549=CARTESIAN_POINT ( 'NONE',  ( -48.73943081701123958, -287.4351093290842414, -345.5413519771897768 ) ) ;
#67550=CARTESIAN_POINT ( 'NONE',  ( 33.59243902203245824, -288.7206532899338640, -250.7722736776322279 ) ) ;
#67552=CARTESIAN_POINT ( 'NONE',  ( 8.088190097750608487, -289.2152523562324404, -327.7085398991985699 ) ) ;
#67553=CARTESIAN_POINT ( 'NONE',  ( -32.10117638658132222, -296.9662699677179489, -345.5468485300314683 ) ) ;
#67555=CARTESIAN_POINT ( 'NONE',  ( 39.20833832427597798, -288.8078325527840775, -274.3866879531319682 ) ) ;
#67556=CARTESIAN_POINT ( 'NONE',  ( -110.0614300989277865, -276.3699032099878536, -290.8831810498074901 ) ) ;
#67557=CARTESIAN_POINT ( 'NONE',  ( -98.78398228410944171, -278.2674287703714526, -316.7572075507293903 ) ) ;
#67558=CARTESIAN_POINT ( 'NONE',  ( -39.58239002344271995, -279.6914903587204435, -193.4018324507144087 ) ) ;
#67559=CARTESIAN_POINT ( 'NONE',  ( 54.16810326369736828, -301.1830605561279413, -195.6852559060315855 ) ) ;
#67560=CARTESIAN_POINT ( 'NONE',  ( -57.91931973830251934, -283.7863288936917456, -198.1852125603847412 ) ) ;
#67562=CARTESIAN_POINT ( 'NONE',  ( -6.230496755101428086, -278.6048701084087043, -202.9457673104903392 ) ) ;
#67563=CARTESIAN_POINT ( 'NONE',  ( -22.15647361619059907, -280.8574611639105001, -343.8077621636666663 ) ) ;
#67565=CARTESIAN_POINT ( 'NONE',  ( -45.59405117923598993, -275.6346754299837585, -346.2728215737361097 ) ) ;
#67566=CARTESIAN_POINT ( 'NONE',  ( -109.5603440661601979, -297.8797707072158687, -285.0927333549785203 ) ) ;
#67567=CARTESIAN_POINT ( 'NONE',  ( 33.27590120156828135, -280.8562369823500831, -300.4073268444819860 ) ) ;
#67568=CARTESIAN_POINT ( 'NONE',  ( -108.4061707829266368, -297.7268255583422842, -252.6108878092626071 ) ) ;
#67569=CARTESIAN_POINT ( 'NONE',  ( -54.50094873605787171, -299.1512974505319562, -195.8033654773533954 ) ) ;
#67570=CARTESIAN_POINT ( 'NONE',  ( -43.47967123505004139, -273.6393426889883358, -197.5476769053416035 ) ) ;
#67571=CARTESIAN_POINT ( 'NONE',  ( 37.61950827621697613, -295.5213466823255999, -267.9490897163788645 ) ) ;
#67572=CARTESIAN_POINT ( 'NONE',  ( 5.177907832212098604, -286.7763733076425297, -206.1019507667887751 ) ) ;
#67574=CARTESIAN_POINT ( 'NONE',  ( -9.371004730146431427, -278.4947637660196733, -200.1688506196131243 ) ) ;
#67575=CARTESIAN_POINT ( 'NONE',  ( -85.16633719142839709, -289.5248581508267307, -330.7765100054237450 ) ) ;
#67576=CARTESIAN_POINT ( 'NONE',  ( -58.76938580649515131, -288.3948114037650043, -340.4445367884876532 ) ) ;
#67577=CARTESIAN_POINT ( 'NONE',  ( 19.80355957313269855, -290.8794933502741742, -221.7676286452262673 ) ) ;
#67579=CARTESIAN_POINT ( 'NONE',  ( -111.8439089875458023, -277.9397250554267202, -284.5643135594219189 ) ) ;
#67580=CARTESIAN_POINT ( 'NONE',  ( 22.79699308962910465, -287.6374045630566911, -311.8720338318446466 ) ) ;
#67582=CARTESIAN_POINT ( 'NONE',  ( -113.6686307448715354, -285.3907036865959981, -278.5476847368751123 ) ) ;
#67583=CARTESIAN_POINT ( 'NONE',  ( -16.67839454482242800, -291.3715271518904046, -196.4297442991912703 ) ) ;
#67584=CARTESIAN_POINT ( 'NONE',  ( -10.85693151091996000, -284.0292260764431944, -342.1938323639706141 ) ) ;
#67585=CARTESIAN_POINT ( 'NONE',  ( -94.28634578134034427, -283.7397928423224585, -316.0571172866168581 ) ) ;
#67586=CARTESIAN_POINT ( 'NONE',  ( -113.6017603480666622, -296.6865266288299381, -259.6166450812182234 ) ) ;
#67587=CARTESIAN_POINT ( 'NONE',  ( 5.450382169254740283, -275.9599185819160425, -210.5480728740110123 ) ) ;
#67588=CARTESIAN_POINT ( 'NONE',  ( -64.65039993833117649, -289.7139660385084881, -200.8772762663025730 ) ) ;
#67589=CARTESIAN_POINT ( 'NONE',  ( 5.420477099717874836, -273.4400744687562224, -210.6449038828786513 ) ) ;
#67592=CARTESIAN_POINT ( 'NONE',  ( 19.75075446432490978, -288.8071609049449648, -222.5734352522242716 ) ) ;
#67594=CARTESIAN_POINT ( 'NONE',  ( -30.60435705395638095, -296.0485136181760026, -346.7554942018302313 ) ) ;
#67595=CARTESIAN_POINT ( 'NONE',  ( -91.60244749309605083, -285.9048202018308302, -221.3003633134682104 ) ) ;
#67597=CARTESIAN_POINT ( 'NONE',  ( 22.45016307081918328, -275.2583318846948828, -318.5249561735231509 ) ) ;
#67598=CARTESIAN_POINT ( 'NONE',  ( 36.98192300237801788, -293.9556352588261348, -250.5793500093642763 ) ) ;
#67599=CARTESIAN_POINT ( 'NONE',  ( 35.94352342945006740, -285.9363108606283390, -289.5856203459081257 ) ) ;
#67600=CARTESIAN_POINT ( 'NONE',  ( 29.55839593848838476, -294.3813002014196059, -308.5492689074562236 ) ) ;
#67601=CARTESIAN_POINT ( 'NONE',  ( -107.7734021145991079, -291.1399995802161698, -251.0877466605860207 ) ) ;
#67604=CARTESIAN_POINT ( 'NONE',  ( -55.03721977837319201, -169.7685131377856180, -360.6694990503212352 ) ) ;
#67605=CARTESIAN_POINT ( 'NONE',  ( -104.8280314947001841, -286.5375332614957529, -234.6346883513537875 ) ) ;
#67606=CARTESIAN_POINT ( 'NONE',  ( 36.57525178469694538, -273.4809262143061233, -305.9938812882205070 ) ) ;
#67608=CARTESIAN_POINT ( 'NONE',  ( -93.66836427075458005, -282.8095319023058209, -317.2816143682121606 ) ) ;
#67609=CARTESIAN_POINT ( 'NONE',  ( -93.32153504367020957, -277.4965134882685334, -323.2770141679658877 ) ) ;
#67610=CARTESIAN_POINT ( 'NONE',  ( 36.36862586835917455, -283.3861069338970538, -257.4453806916467329 ) ) ;
#67611=CARTESIAN_POINT ( 'NONE',  ( -92.99569426845059184, -240.8231148737314413, -340.8140838316123222 ) ) ;
#67612=CARTESIAN_POINT ( 'NONE',  ( 1.776775480513330452, -281.1143465880900862, -335.9991493262335780 ) ) ;
#67613=CARTESIAN_POINT ( 'NONE',  ( 17.19299240869666079, -284.8550474041055622, -219.3734922805081169 ) ) ;
#67614=CARTESIAN_POINT ( 'NONE',  ( -43.95887525711700761, -275.8298985963662631, -194.8333803553555015 ) ) ;
#67615=CARTESIAN_POINT ( 'NONE',  ( -9.201388971772328063, -295.1664038117265818, -337.7995927981606314 ) ) ;
#67616=CARTESIAN_POINT ( 'NONE',  ( 35.78780539544837325, -292.1348332891051882, -262.5661422521280315 ) ) ;
#67617=CARTESIAN_POINT ( 'NONE',  ( -107.3297964742374688, -279.6127572436719220, -238.3741459667424465 ) ) ;
#67618=CARTESIAN_POINT ( 'NONE',  ( 9.664048229737067786, -276.3838701438514818, -326.2132407830538909 ) ) ;
#67619=CARTESIAN_POINT ( 'NONE',  ( 37.91806818040716109, -274.2873166390560868, -255.6146002645775468 ) ) ;
#67621=CARTESIAN_POINT ( 'NONE',  ( 36.24934055300464308, -273.7386169413551897, -284.8957898882777613 ) ) ;
#67623=CARTESIAN_POINT ( 'NONE',  ( -24.98507369733978223, -296.3229290802827336, -345.8198119692100363 ) ) ;
#67625=CARTESIAN_POINT ( 'NONE',  ( -70.34180879251273666, -284.5773425291053513, -335.8367380935204665 ) ) ;
#67626=CARTESIAN_POINT ( 'NONE',  ( -30.28636985388002500, -284.7241938046115024, -346.0195367341307247 ) ) ;
#67627=CARTESIAN_POINT ( 'NONE',  ( -30.51351288922421645, -285.4892176662571615, -197.5279116498812186 ) ) ;
#67628=CARTESIAN_POINT ( 'NONE',  ( 31.01136717562667044, -274.3223346835467851, -298.3232246276980391 ) ) ;
#67629=CARTESIAN_POINT ( 'NONE',  ( -67.03219711769824585, -285.3059087430916065, -338.4141686933419351 ) ) ;
#67630=CARTESIAN_POINT ( 'NONE',  ( -21.52288415571240421, -275.3256493941568124, -342.3891024212062462 ) ) ;
#67631=CARTESIAN_POINT ( 'NONE',  ( -80.99246365659742253, -278.7406116943267875, -329.2579508013222949 ) ) ;
#67634=CARTESIAN_POINT ( 'NONE',  ( 39.02110001429821295, -282.2421584506290628, -261.3587114209443030 ) ) ;
#67635=CARTESIAN_POINT ( 'NONE',  ( -48.11637030904267931, -280.4110576700969091, -194.1270470132709249 ) ) ;
#67639=CARTESIAN_POINT ( 'NONE',  ( -4.053772750359502020, -288.3468017202550300, -202.2864160177626047 ) ) ;
#67640=CARTESIAN_POINT ( 'NONE',  ( -103.8611543254021967, -296.1606551595554038, -239.7799996812944130 ) ) ;
#67641=CARTESIAN_POINT ( 'NONE',  ( -68.28013332678875713, -291.0049469301220597, -199.9470114095400390 ) ) ;
#67642=CARTESIAN_POINT ( 'NONE',  ( 30.34278669191611399, -286.1910138262050509, -300.4345436580528599 ) ) ;
#67643=CARTESIAN_POINT ( 'NONE',  ( 22.42976847945794105, -286.7221924786719569, -313.2883407966180584 ) ) ;
#67644=CARTESIAN_POINT ( 'NONE',  ( -64.42178551901656647, -289.9336815404418530, -201.4660300265077808 ) ) ;
#67645=CARTESIAN_POINT ( 'NONE',  ( -89.95815940492823870, -286.4938518603173634, -219.1155312442799357 ) ) ;
#67646=CARTESIAN_POINT ( 'NONE',  ( -79.13344159225331964, -275.6153139123474034, -332.7008608179157250 ) ) ;
#67647=CARTESIAN_POINT ( 'NONE',  ( 38.29388296519224610, -286.0743698888280733, -280.0419751694623756 ) ) ;
#67648=CARTESIAN_POINT ( 'NONE',  ( 18.77296796986961880, -288.8595077083489855, -220.5236111560628558 ) ) ;
#67649=CARTESIAN_POINT ( 'NONE',  ( -96.72723180373841956, -287.9216386109393966, -316.4413421396330364 ) ) ;
#67650=CARTESIAN_POINT ( 'NONE',  ( -32.11699080309450238, -283.9258833961350206, -343.4098062718335882 ) ) ;
#67651=CARTESIAN_POINT ( 'NONE',  ( -68.87779351538624439, -293.6387011420119393, -202.1158679811317995 ) ) ;
#67652=CARTESIAN_POINT ( 'NONE',  ( 82.17447117356790898, -297.5427909045017714, -195.1407487411256341 ) ) ;
#67654=CARTESIAN_POINT ( 'NONE',  ( -40.40679947260564120, -299.9341872900681665, -194.8121571392851479 ) ) ;
#67655=CARTESIAN_POINT ( 'NONE',  ( -35.64883519073631390, -279.2710619372849123, -197.2067988523656936 ) ) ;
#67656=CARTESIAN_POINT ( 'NONE',  ( 37.68878881932509017, -279.5288648190948493, -268.5602934286727077 ) ) ;
#67657=CARTESIAN_POINT ( 'NONE',  ( 32.07973605760906821, -293.1737036938523602, -303.4217676600216009 ) ) ;
#67658=CARTESIAN_POINT ( 'NONE',  ( -95.39375475043335939, -271.4310699340612700, -224.4488868151456415 ) ) ;
#67659=CARTESIAN_POINT ( 'NONE',  ( -3.228936006821487847, -274.6777795793782957, -336.5248053395331453 ) ) ;
#67660=CARTESIAN_POINT ( 'NONE',  ( -71.14280196073748641, -296.8232007806758475, -335.6341335305513667 ) ) ;
#67662=CARTESIAN_POINT ( 'NONE',  ( -91.73677117324264429, -271.8697296988864309, -216.6975126408426604 ) ) ;
#67663=CARTESIAN_POINT ( 'NONE',  ( 36.47025277189471382, -292.0214278169038380, -288.4645845785557299 ) ) ;
#67664=CARTESIAN_POINT ( 'NONE',  ( -2.173684423439532498, -293.9525609186050019, -205.7048296468088040 ) ) ;
#67665=DIRECTION ( 'NONE',  ( -1.000000000000000000, -0.000000000000000000, -0.000000000000000000 ) ) ;
#67666=CARTESIAN_POINT ( 'NONE',  ( 31.69582339886613198, -294.6782662871694924, -294.7290245203899417 ) ) ;
#67668=CARTESIAN_POINT ( 'NONE',  ( -85.08025831850403620, -281.7275247512647525, -328.6658078595815482 ) ) ;
#67669=CARTESIAN_POINT ( 'NONE',  ( -10.49000150794004682, -294.6917916147372694, -338.2432679279846184 ) ) ;
#67670=CARTESIAN_POINT ( 'NONE',  ( -2.892840669931094677, -282.6095478170842625, -339.2399569898188929 ) ) ;
#67671=CARTESIAN_POINT ( 'NONE',  ( -12.01548698114655878, -282.2992288453663718, -199.1170261378642294 ) ) ;
#67672=CARTESIAN_POINT ( 'NONE',  ( -110.9045639273811474, -284.5057726810414920, -247.5046716233837003 ) ) ;
#67673=CARTESIAN_POINT ( 'NONE',  ( -91.11647521756077595, -289.2856518755714319, -218.3197691319824116 ) ) ;
#67674=CARTESIAN_POINT ( 'NONE',  ( 37.18415559740575560, -280.2396289614213742, -286.8105527711588820 ) ) ;
#67675=CARTESIAN_POINT ( 'NONE',  ( -49.48664179749899716, -284.5790291060191066, -197.8265591579031195 ) ) ;
#67676=CARTESIAN_POINT ( 'NONE',  ( 16.45926741141646943, -287.2299039735248130, -325.0879318871068904 ) ) ;
#67678=CARTESIAN_POINT ( 'NONE',  ( 12.91441070691149662, -295.9369819510189359, -324.4752687276510983 ) ) ;
#67679=CARTESIAN_POINT ( 'NONE',  ( -113.4902521127258836, -279.8900259178460033, -277.2958018919841834 ) ) ;
#67680=CARTESIAN_POINT ( 'NONE',  ( 29.43293115384220826, -292.0326663717503379, -305.2832516094761104 ) ) ;
#67681=CARTESIAN_POINT ( 'NONE',  ( -64.82013868644347099, -279.3498227320561682, -202.7074196268862920 ) ) ;
#67682=CARTESIAN_POINT ( 'NONE',  ( 38.60663593945798766, -293.8784451657110139, -283.1236972015734068 ) ) ;
#67683=CARTESIAN_POINT ( 'NONE',  ( -111.5787022373148858, -282.8148365000241142, -256.0116569892018674 ) ) ;
#67684=CARTESIAN_POINT ( 'NONE',  ( -79.09116339031255905, -279.6149906452071718, -332.7291837752894139 ) ) ;
#67685=CARTESIAN_POINT ( 'NONE',  ( -0.6504171600917483254, -293.6109337637079761, -333.8000482619797253 ) ) ;
#67686=CARTESIAN_POINT ( 'NONE',  ( -4.479461041248472775, -296.4633562459687255, -195.3723136117041292 ) ) ;
#67689=CARTESIAN_POINT ( 'NONE',  ( 37.07085638919105719, -283.6160204865634569, -276.8700250130047493 ) ) ;
#67690=CARTESIAN_POINT ( 'NONE',  ( -109.1049325678878006, -296.2414166074379409, -256.5822255039538504 ) ) ;
#67692=CARTESIAN_POINT ( 'NONE',  ( 31.98288692825983404, -278.6237833571634610, -237.0123917617631264 ) ) ;
#67693=CARTESIAN_POINT ( 'NONE',  ( -3.527245894643499469, -297.5245468185709115, -193.6016564146562473 ) ) ;
#67694=CARTESIAN_POINT ( 'NONE',  ( 35.37504116671787102, -288.5642618076058170, -246.4100107637281099 ) ) ;
#67695=CARTESIAN_POINT ( 'NONE',  ( -69.97436101230287875, -289.3277194220793263, -335.6751262217861722 ) ) ;
#67696=CARTESIAN_POINT ( 'NONE',  ( -37.02459026532761754, -281.5763177061006672, -196.6684643728150945 ) ) ;
#67697=CARTESIAN_POINT ( 'NONE',  ( -65.98529596308397061, -299.4322596722847152, -202.1151039421012001 ) ) ;
#67698=CARTESIAN_POINT ( 'NONE',  ( -35.63828123159275663, -278.8688838506628258, -196.9713430945191703 ) ) ;
#67699=EDGE_LOOP ( 'NONE', ( #70324, #69808 ) ) ;
#67700=CARTESIAN_POINT ( 'NONE',  ( -68.16509163271760485, -297.3251750284244395, -199.7659592282151948 ) ) ;
#67701=CARTESIAN_POINT ( 'NONE',  ( -41.70114407029316084, -293.9171053130156110, -195.9980460610264856 ) ) ;
#67703=CARTESIAN_POINT ( 'NONE',  ( -72.40046885151168965, -290.1806441474411713, -334.5076331176156259 ) ) ;
#67706=CARTESIAN_POINT ( 'NONE',  ( 3.496032565038655893, -290.7341866847588108, -206.4821110034023093 ) ) ;
#67707=CARTESIAN_POINT ( 'NONE',  ( -81.95368129959769021, -297.0918911847159620, -212.4882258021241341 ) ) ;
#67709=CARTESIAN_POINT ( 'NONE',  ( -101.7059337997187356, -291.5289943852437773, -311.4455487226369996 ) ) ;
#67710=CARTESIAN_POINT ( 'NONE',  ( -111.2869819898779866, -287.4805209788416391, -234.7871824221999191 ) ) ;
#67711=CARTESIAN_POINT ( 'NONE',  ( 33.56992404336133973, -289.2424871895032084, -246.4535881379001410 ) ) ;
#67712=CARTESIAN_POINT ( 'NONE',  ( -3.049479776392111319, -274.5977860927958432, -336.8748162184514854 ) ) ;
#67713=CARTESIAN_POINT ( 'NONE',  ( 34.90088029841781037, -277.2399738718721096, -252.4077401820034652 ) ) ;
#67714=CARTESIAN_POINT ( 'NONE',  ( -60.68783329882943178, -289.8268926802805368, -199.6227246393132475 ) ) ;
#67715=CARTESIAN_POINT ( 'NONE',  ( -94.98176857742367929, -281.0867563655821186, -221.1687522319337234 ) ) ;
#67716=ORIENTED_EDGE ( 'NONE', *, *, #48099, .T. ) ;
#67717=CARTESIAN_POINT ( 'NONE',  ( -36.20024906065894044, -282.3860513726920090, -343.4541392499589278 ) ) ;
#67718=CARTESIAN_POINT ( 'NONE',  ( -111.8715035675152762, -279.4041299241476963, -288.4937178898858861 ) ) ;
#67719=CARTESIAN_POINT ( 'NONE',  ( 16.95256563256307913, -279.5994343103488973, -216.2483896918401172 ) ) ;
#67720=CARTESIAN_POINT ( 'NONE',  ( -1.422236905112849836, -275.4579193733644047, -202.5185621987752995 ) ) ;
#67724=CARTESIAN_POINT ( 'NONE',  ( -64.67001702453850953, -275.2218596178875032, -199.1019123151973247 ) ) ;
#67725=CARTESIAN_POINT ( 'NONE',  ( -21.39648532958013050, -276.7662352645559167, -200.3538533559491555 ) ) ;
#67728=CARTESIAN_POINT ( 'NONE',  ( -112.2375992108470228, -298.5015950462242245, -274.3114276736488932 ) ) ;
#67729=CARTESIAN_POINT ( 'NONE',  ( -90.80882447132154311, -290.9124185237738516, -320.5899216834986873 ) ) ;
#67730=CARTESIAN_POINT ( 'NONE',  ( -54.25397744942461742, -291.0264746411680790, -344.4957981948597876 ) ) ;
#67731=CARTESIAN_POINT ( 'NONE',  ( 11.00442705175344749, -292.0906104290316989, -215.4615969200426946 ) ) ;
#67732=CARTESIAN_POINT ( 'NONE',  ( 31.36965327955490324, -286.6140204605208623, -235.7449827859915956 ) ) ;
#67734=CARTESIAN_POINT ( 'NONE',  ( -36.20138663600549478, -281.4374897226920211, -344.1523105634200874 ) ) ;
#67735=CARTESIAN_POINT ( 'NONE',  ( 21.34835292803084528, -290.0422959739304360, -315.8387562628982437 ) ) ;
#67736=CARTESIAN_POINT ( 'NONE',  ( -89.39763245738217279, -282.2811429183595351, -322.5948919052556221 ) ) ;
#67737=CARTESIAN_POINT ( 'NONE',  ( -7.816595296067766263, -281.7625141631157817, -203.0457080379315187 ) ) ;
#67738=CARTESIAN_POINT ( 'NONE',  ( 23.96156132175256559, -289.1105069894522330, -316.5642601842934027 ) ) ;
#67739=CARTESIAN_POINT ( 'NONE',  ( -96.45918423570998357, -279.6448127014732563, -227.4296433448164123 ) ) ;
#67740=CARTESIAN_POINT ( 'NONE',  ( 15.17715963397304435, -291.5684594889823984, -214.5228877008711947 ) ) ;
#67741=CARTESIAN_POINT ( 'NONE',  ( 28.55479088422166001, -287.8373407107815751, -230.7387650182011782 ) ) ;
#67742=CARTESIAN_POINT ( 'NONE',  ( -18.20340191925394890, -286.7846169262814442, -195.7859127869537872 ) ) ;
#67743=CARTESIAN_POINT ( 'NONE',  ( -90.74001278311652641, -284.0030235207151463, -320.1368169741696192 ) ) ;
#67746=CARTESIAN_POINT ( 'NONE',  ( 14.57425130791220980, -294.6334574806179489, -215.1072283240156651 ) ) ;
#67747=CARTESIAN_POINT ( 'NONE',  ( 37.29908086244962107, -292.4491193489233183, -287.2145997093907113 ) ) ;
#67748=CARTESIAN_POINT ( 'NONE',  ( -24.29943660481183798, -275.9404235108585226, -342.4773420176054515 ) ) ;
#67749=CARTESIAN_POINT ( 'NONE',  ( -113.2875645272479801, -296.0528614967237218, -258.2138243589183730 ) ) ;
#67750=CARTESIAN_POINT ( 'NONE',  ( 17.26484732444187387, -291.3289833482157292, -220.8005691610107135 ) ) ;
#67751=CARTESIAN_POINT ( 'NONE',  ( -103.4271690398474988, -295.2395170403725615, -236.9201329468618837 ) ) ;
#67752=CARTESIAN_POINT ( 'NONE',  ( -55.12332557170220326, -293.0234003247683177, -199.1505548600890165 ) ) ;
#67753=CARTESIAN_POINT ( 'NONE',  ( 4.669580318944723807, -293.7135962120383397, -210.2216279416927307 ) ) ;
#67755=CARTESIAN_POINT ( 'NONE',  ( 7.784699692153664863, -292.4373024797957896, -330.4746477644270044 ) ) ;
#67756=CARTESIAN_POINT ( 'NONE',  ( -112.3912264470853870, -298.5590368601372120, -269.8377770872875203 ) ) ;
#67757=CARTESIAN_POINT ( 'NONE',  ( 22.15983908085178555, -289.0883344423215817, -313.0574325810163714 ) ) ;
#67758=CARTESIAN_POINT ( 'NONE',  ( -48.23084345033734621, -279.1698128255303004, -344.9781490221671447 ) ) ;
#67759=CARTESIAN_POINT ( 'NONE',  ( -23.02822260613217864, -275.6680284131264784, -345.6688129934878475 ) ) ;
#67760=CARTESIAN_POINT ( 'NONE',  ( -93.09254255074064588, -272.6257236916284796, -217.3781776140207285 ) ) ;
#67761=CARTESIAN_POINT ( 'NONE',  ( 36.12078151329666298, -279.7875446359871603, -282.3851767820270879 ) ) ;
#67762=CARTESIAN_POINT ( 'NONE',  ( -31.53180984173248191, -275.3799670801577122, -346.3913862438355409 ) ) ;
#67763=CARTESIAN_POINT ( 'NONE',  ( -102.9651863840894208, -295.6844126480182240, -237.1600709593430736 ) ) ;
#67765=CARTESIAN_POINT ( 'NONE',  ( -108.6361481453368043, -273.4163851998842460, -254.2057984095889651 ) ) ;
#67767=CARTESIAN_POINT ( 'NONE',  ( -99.34195973377948974, -287.9943343305151302, -313.1907177047527284 ) ) ;
#67768=CARTESIAN_POINT ( 'NONE',  ( -46.17667554310626343, -273.7702700978575194, -197.8977257495770061 ) ) ;
#67769=CARTESIAN_POINT ( 'NONE',  ( -26.14455805463359539, -288.9133496689164531, -346.5426381130156415 ) ) ;
#67770=CARTESIAN_POINT ( 'NONE',  ( -54.25112652680952152, -299.8159086578167489, -196.9276235907035186 ) ) ;
#67771=CARTESIAN_POINT ( 'NONE',  ( -109.2132195524827267, -294.8209521526893582, -249.5161396050932012 ) ) ;
#67772=CARTESIAN_POINT ( 'NONE',  ( -33.07794900383075287, -282.1969327789103659, -347.0943613475226357 ) ) ;
#67774=CARTESIAN_POINT ( 'NONE',  ( 9.489684339936221846, -280.4085116167094611, -329.0085771338789300 ) ) ;
#67776=CARTESIAN_POINT ( 'NONE',  ( -108.1308130345192495, -289.6018912881219194, -250.9695734453144098 ) ) ;
#67777=CARTESIAN_POINT ( 'NONE',  ( -26.58684975546040619, -281.0536038529025973, -343.8652996948007967 ) ) ;
#67780=CARTESIAN_POINT ( 'NONE',  ( -55.47182832744906733, -289.8186799491717238, -197.5854414335602200 ) ) ;
#67781=CARTESIAN_POINT ( 'NONE',  ( -46.28190640407311918, -275.4568002816404260, -197.2120888475302820 ) ) ;
#67782=CARTESIAN_POINT ( 'NONE',  ( -21.79152322614257287, -284.0621815175651932, -345.3691223273917217 ) ) ;
#67783=CARTESIAN_POINT ( 'NONE',  ( -78.04487814606238771, -271.5894186498043155, -206.7013544275120864 ) ) ;
#67784=CARTESIAN_POINT ( 'NONE',  ( -65.31569641794466463, -283.4282414377342434, -337.8021258867885876 ) ) ;
#67785=CARTESIAN_POINT ( 'NONE',  ( 32.61634727392659272, -276.6749586450051765, -247.3664955464804223 ) ) ;
#67786=CARTESIAN_POINT ( 'NONE',  ( -40.50253187497059315, -277.8957125937656087, -343.4667756798746154 ) ) ;
#67788=CARTESIAN_POINT ( 'NONE',  ( -33.14452843634265378, -284.9994731462925870, -345.2563822137155398 ) ) ;
#67791=CARTESIAN_POINT ( 'NONE',  ( -112.3417001281054723, -270.5523139186827279, -270.3356821209761165 ) ) ;
#67792=CARTESIAN_POINT ( 'NONE',  ( -0.7080456332996576396, -294.4126420152652486, -338.1032159629180569 ) ) ;
#67793=CARTESIAN_POINT ( 'NONE',  ( -33.17142365197523191, -288.0846860420366511, -195.7819544807134378 ) ) ;
#67794=FACE_OUTER_BOUND ( 'NONE', #57397, .T. ) ;
#67795=CARTESIAN_POINT ( 'NONE',  ( -37.37352853689063181, -286.5523547857346784, -350.3611179825600175 ) ) ;
#67796=CARTESIAN_POINT ( 'NONE',  ( -114.0682601330215107, -277.4930007894196251, -268.7270557508198294 ) ) ;
#67797=CARTESIAN_POINT ( 'NONE',  ( -107.6213552519863583, -289.3305374004335704, -240.9126801753092479 ) ) ;
#67798=CARTESIAN_POINT ( 'NONE',  ( -108.0517734583732761, -285.7997242717115682, -291.1616919183630330 ) ) ;
#67799=CARTESIAN_POINT ( 'NONE',  ( -94.37272237598270408, -279.6524442625789106, -317.5554998544593559 ) ) ;
#67800=CARTESIAN_POINT ( 'NONE',  ( -65.67586712538583527, -287.1140455144932275, -199.3838312484235757 ) ) ;
#67801=CARTESIAN_POINT ( 'NONE',  ( -37.52039300842150027, -285.0545814174431598, -345.3736788903798924 ) ) ;
#67802=CARTESIAN_POINT ( 'NONE',  ( -34.28897043574578163, -277.1814415574908139, -347.3005801976481735 ) ) ;
#67803=CARTESIAN_POINT ( 'NONE',  ( 10.26600815775594633, -296.6710508435074303, -195.7324710267420755 ) ) ;
#67804=CARTESIAN_POINT ( 'NONE',  ( -25.39349840143035664, -280.0337503176937730, -194.2937762386257532 ) ) ;
#67805=CARTESIAN_POINT ( 'NONE',  ( -94.73925213247066779, -299.1314114095068817, -222.9404875693416557 ) ) ;
#67807=CARTESIAN_POINT ( 'NONE',  ( -37.37352853689063892, -276.5519495502701943, -195.3611179825600175 ) ) ;
#67808=CARTESIAN_POINT ( 'NONE',  ( -112.5381433073586805, -270.9350727805710335, -259.0727742121037522 ) ) ;
#67810=CARTESIAN_POINT ( 'NONE',  ( -41.86665514001207811, -276.6183232892640262, -343.2950060033076056 ) ) ;
#67811=CARTESIAN_POINT ( 'NONE',  ( -66.09250230434403761, -274.8892274802209386, -199.3442019789883375 ) ) ;
#67812=CARTESIAN_POINT ( 'NONE',  ( 15.58261763641016806, -281.3838802044789418, -325.9654056018807751 ) ) ;
#67813=CARTESIAN_POINT ( 'NONE',  ( -7.793618437226421669, -290.4198249741118047, -338.2752188013716363 ) ) ;
#67814=CARTESIAN_POINT ( 'NONE',  ( -109.6822048469219908, -297.7637299367515880, -294.6419567075516852 ) ) ;
#67815=CARTESIAN_POINT ( 'NONE',  ( -69.34795967050554566, -296.6690523070229233, -339.9715099452233744 ) ) ;
#67816=CARTESIAN_POINT ( 'NONE',  ( -5.278652740791745401, -294.4751928973149688, -202.7305049653961362 ) ) ;
#67817=CARTESIAN_POINT ( 'NONE',  ( 4.392047730498685354, -280.4881251823759385, -332.5391834806800375 ) ) ;
#67818=CARTESIAN_POINT ( 'NONE',  ( -49.39876358561404146, -281.8174174048526197, -196.9040460542461233 ) ) ;
#67819=CARTESIAN_POINT ( 'NONE',  ( -111.9855616574490824, -270.6085108309786733, -267.5507348244821060 ) ) ;
#67820=CARTESIAN_POINT ( 'NONE',  ( -97.40116728422712811, -285.5190525078500627, -317.2578217399354230 ) ) ;
#67821=CARTESIAN_POINT ( 'NONE',  ( 15.26083122062464703, -285.7373727780189370, -219.3003721083325956 ) ) ;
#67822=CARTESIAN_POINT ( 'NONE',  ( 23.67150155679529178, -280.2753533880368195, -223.5346683830870234 ) ) ;
#67823=CARTESIAN_POINT ( 'NONE',  ( -76.02243030850807770, -209.4518847369260754, -356.5868710737057086 ) ) ;
#67825=CARTESIAN_POINT ( 'NONE',  ( 21.93644909056341064, -286.7789687740857403, -318.5969222939634733 ) ) ;
#67826=CARTESIAN_POINT ( 'NONE',  ( -42.67143833779803686, -285.6498094414148454, -197.5221104102778895 ) ) ;
#67828=CARTESIAN_POINT ( 'NONE',  ( -97.79224851240952887, -284.9986797636298661, -317.5545890481214428 ) ) ;
#67829=CARTESIAN_POINT ( 'NONE',  ( 28.05132950365664612, -276.3272678145984855, -302.9687985350306576 ) ) ;
#67830=CARTESIAN_POINT ( 'NONE',  ( -90.56149097500754408, -290.2400402312915162, -215.0683518601522621 ) ) ;
#67831=CARTESIAN_POINT ( 'NONE',  ( 33.07627213693600510, -281.8090052431759318, -239.4641607154334793 ) ) ;
#67833=CARTESIAN_POINT ( 'NONE',  ( -108.9622107912893512, -280.4097785535952880, -243.8795769879390889 ) ) ;
#67834=CARTESIAN_POINT ( 'NONE',  ( 33.15188035396288058, -281.4909244181411054, -239.4354101933971037 ) ) ;
#67835=CARTESIAN_POINT ( 'NONE',  ( -92.05005921254146983, -288.6952119285918457, -226.6919474004047572 ) ) ;
#67836=CARTESIAN_POINT ( 'NONE',  ( 26.08411754451436693, -23.25919466593375873, -345.2244097993914806 ) ) ;
#67838=CARTESIAN_POINT ( 'NONE',  ( -18.53213648314174122, -278.8094562997310959, -342.7919728649139870 ) ) ;
#67839=CARTESIAN_POINT ( 'NONE',  ( -104.8592795955056118, -255.4662412201343500, -326.3873165879509770 ) ) ;
#67840=CARTESIAN_POINT ( 'NONE',  ( 17.00650590315697031, -280.2933951682540510, -321.6032218939701579 ) ) ;
#67841=CARTESIAN_POINT ( 'NONE',  ( -39.16256298938664315, -297.3773215372942786, -197.2694392661224185 ) ) ;
#67842=CARTESIAN_POINT ( 'NONE',  ( 25.66065556470347531, -293.6444961109544920, -314.5455173815605576 ) ) ;
#67843=CARTESIAN_POINT ( 'NONE',  ( -76.15440596507517057, -208.4761271767036419, -353.6627180100991268 ) ) ;
#67844=CARTESIAN_POINT ( 'NONE',  ( -111.3369717193388908, -271.4842549895164439, -250.7163547451768295 ) ) ;
#67845=CARTESIAN_POINT ( 'NONE',  ( -75.14298698906080176, -287.9647261292154212, -333.7597444371619417 ) ) ;
#67846=CARTESIAN_POINT ( 'NONE',  ( -34.22603441533227198, -296.8729777861386765, -344.5309104142584147 ) ) ;
#67847=CARTESIAN_POINT ( 'NONE',  ( -37.29727805885298153, -287.3678590389684473, -196.8554559647179190 ) ) ;
#67849=CARTESIAN_POINT ( 'NONE',  ( -2.174344376177569149, -293.4473542348166006, -202.1109315974390199 ) ) ;
#67850=CARTESIAN_POINT ( 'NONE',  ( -108.4837844942666010, -284.8245598614978462, -287.0528345518507649 ) ) ;
#67851=CARTESIAN_POINT ( 'NONE',  ( -29.09726686348604119, -296.9481435779741219, -193.7598320506033929 ) ) ;
#67852=CARTESIAN_POINT ( 'NONE',  ( -19.43435153304433882, -293.0795312831044725, -195.5836872514845197 ) ) ;
#67854=CARTESIAN_POINT ( 'NONE',  ( -30.70882872728190094, -292.6260867691669318, -193.6563834882051935 ) ) ;
#67855=CARTESIAN_POINT ( 'NONE',  ( -106.9514523044458087, -290.4253601445953450, -292.5165272901649018 ) ) ;
#67858=CARTESIAN_POINT ( 'NONE',  ( -34.13637962752525112, -299.9522818879969464, -194.5953074871426338 ) ) ;
#67859=CARTESIAN_POINT ( 'NONE',  ( -76.21790563120529782, -272.3399534283387311, -204.2949139669707677 ) ) ;
#67861=CARTESIAN_POINT ( 'NONE',  ( 1.215027249381221086, -281.5826070308897329, -332.6841806656848917 ) ) ;
#67863=CARTESIAN_POINT ( 'NONE',  ( -77.78789002591544488, -277.0872178091924525, -335.8724981378930465 ) ) ;
#67865=CARTESIAN_POINT ( 'NONE',  ( -102.7299144268593096, -271.4139592284410583, -236.0332178671868633 ) ) ;
#67866=CARTESIAN_POINT ( 'NONE',  ( -97.41904388694345585, -281.0126603772627618, -226.7540285483705418 ) ) ;
#67867=CARTESIAN_POINT ( 'NONE',  ( 33.26583397292183975, -273.9908022776962753, -293.2836311160724563 ) ) ;
#67868=CARTESIAN_POINT ( 'NONE',  ( -106.3553288552089668, -297.4244227226124622, -295.4954613460365636 ) ) ;
#67869=CARTESIAN_POINT ( 'NONE',  ( -72.02972481751037037, -274.5231957475813260, -205.8053883274620830 ) ) ;
#67870=CARTESIAN_POINT ( 'NONE',  ( -82.51290234280770619, -299.0471689013976402, -208.9277779076990953 ) ) ;
#67871=CARTESIAN_POINT ( 'NONE',  ( 23.17436010557835502, -272.9622424397318809, -225.4588545732813714 ) ) ;
#67872=CARTESIAN_POINT ( 'NONE',  ( 34.58197312765408782, -294.0304501379856674, -257.2195276941404813 ) ) ;
#67873=CARTESIAN_POINT ( 'NONE',  ( -14.64758602862610992, -290.9268476257366842, -200.3586030174679138 ) ) ;
#67874=DIRECTION ( 'NONE',  ( 0.000000000000000000, 0.000000000000000000, 1.000000000000000000 ) ) ;
#67875=CARTESIAN_POINT ( 'NONE',  ( -22.94426238458952483, -277.3651781578207647, -345.9946271480175142 ) ) ;
#67876=CARTESIAN_POINT ( 'NONE',  ( -54.21359685667891171, -273.9960433975784895, -199.3376070494722967 ) ) ;
#67877=CARTESIAN_POINT ( 'NONE',  ( 23.00354655200976595, -280.8695673351771802, -317.4115236475249162 ) ) ;
#67878=CARTESIAN_POINT ( 'NONE',  ( 36.55959091783275028, -295.7291575834854029, -284.1649664084121696 ) ) ;
#67880=CARTESIAN_POINT ( 'NONE',  ( -108.5202381618143050, -283.9726576883808207, -253.3892338750122235 ) ) ;
#67881=CARTESIAN_POINT ( 'NONE',  ( -109.7328760552722287, -282.2922277438636911, -290.5983627637394875 ) ) ;
#67882=CARTESIAN_POINT ( 'NONE',  ( 23.55001489868414666, -273.5565685099415418, -229.0157055706463893 ) ) ;
#67883=CARTESIAN_POINT ( 'NONE',  ( 35.73046154822215215, -283.3347252669242380, -253.4097918303002075 ) ) ;
#67887=CARTESIAN_POINT ( 'NONE',  ( -96.30394343284984870, -271.6071262299524847, -222.0717842561393525 ) ) ;
#67888=CARTESIAN_POINT ( 'NONE',  ( -74.40939965479820728, -279.5441218691685776, -335.7523565334744831 ) ) ;
#67890=CARTESIAN_POINT ( 'NONE',  ( -26.84578467067315444, -288.1046494482942535, -195.4811529616483483 ) ) ;
#67892=CARTESIAN_POINT ( 'NONE',  ( -72.57218199827893557, -287.5183519005814787, -336.5857462262574700 ) ) ;
#67893=DIRECTION ( 'NONE',  ( 0.000000000000000000, 0.000000000000000000, 1.000000000000000000 ) ) ;
#67894=CARTESIAN_POINT ( 'NONE',  ( -104.0732405473320483, -295.7584767285530916, -239.6769061020408174 ) ) ;
#67895=CARTESIAN_POINT ( 'NONE',  ( -0.3969470701810811075, -286.6954378144469615, -334.8093351585907840 ) ) ;
#67896=CARTESIAN_POINT ( 'NONE',  ( 133.9787772367566561, 181.9811788097603937, -239.6702418147338562 ) ) ;
#67897=CARTESIAN_POINT ( 'NONE',  ( -98.83747485365626062, -293.9693470199541707, -313.2944423443192932 ) ) ;
#67898=CARTESIAN_POINT ( 'NONE',  ( 26.56774214911342114, -285.4793481802478823, -228.6683015739363043 ) ) ;
#67899=CARTESIAN_POINT ( 'NONE',  ( 35.93663529450428484, -283.2720286767190601, -279.5377115546359050 ) ) ;
#67900=CARTESIAN_POINT ( 'NONE',  ( -5.895603417133877144, -280.8842764895841242, -339.5356582282058753 ) ) ;
#67901=CARTESIAN_POINT ( 'NONE',  ( -78.17441562460498972, -289.6179411365828287, -330.9338669709941314 ) ) ;
#67902=CARTESIAN_POINT ( 'NONE',  ( -4.097492321258143555, -281.9246379407643417, -204.6950212470591453 ) ) ;
#67903=CARTESIAN_POINT ( 'NONE',  ( 25.70335987136919087, -282.8649091829875033, -307.5816233393840662 ) ) ;
#67904=CARTESIAN_POINT ( 'NONE',  ( 11.37215196813228069, -290.3605622479366275, -327.8534428077932716 ) ) ;
#67905=CARTESIAN_POINT ( 'NONE',  ( -113.8421273244509280, -272.9926298029299119, -261.7920497570210046 ) ) ;
#67906=CARTESIAN_POINT ( 'NONE',  ( -94.14526433434653541, -273.2593801714742199, -218.3574691540785579 ) ) ;
#67907=CARTESIAN_POINT ( 'NONE',  ( -41.71383107583249483, -293.9768337946600241, -195.7934981620775261 ) ) ;
#67909=CARTESIAN_POINT ( 'NONE',  ( 35.78497577281001440, -284.2662352645559167, -287.0191576251351080 ) ) ;
#67911=CARTESIAN_POINT ( 'NONE',  ( 36.92034388086303665, -273.7051210497410239, -282.3136704404327020 ) ) ;
#67914=CARTESIAN_POINT ( 'NONE',  ( -103.1485327335104500, -295.4583696193757305, -231.8397191248259617 ) ) ;
#67915=CARTESIAN_POINT ( 'NONE',  ( -105.8481477381913578, -291.7872890314100687, -297.9446155939880327 ) ) ;
#67916=CARTESIAN_POINT ( 'NONE',  ( -8.923555251079450912, -273.7824066312638251, -202.9550551376902376 ) ) ;
#67917=CARTESIAN_POINT ( 'NONE',  ( -96.31160387745562446, -291.4574693901413411, -314.5778509817639588 ) ) ;
#67918=CARTESIAN_POINT ( 'NONE',  ( -75.11119822966473691, -292.4771540352930401, -207.5573976376408893 ) ) ;
#67919=CARTESIAN_POINT ( 'NONE',  ( -48.45907662313171471, -284.9557535613526511, -343.5347331148200851 ) ) ;
#67920=CARTESIAN_POINT ( 'NONE',  ( -64.19883188903861537, -293.1339156866479811, -198.7700573036570120 ) ) ;
#67921=CARTESIAN_POINT ( 'NONE',  ( -39.21650298078071728, -293.3442860848596752, -193.8642898326153272 ) ) ;
#67922=CARTESIAN_POINT ( 'NONE',  ( 24.42612397261670765, -293.9240514454459685, -309.3628266954221431 ) ) ;
#67923=CARTESIAN_POINT ( 'NONE',  ( 0.02656974400907759562, -290.5553912152586236, -335.4486944531389554 ) ) ;
#67924=CARTESIAN_POINT ( 'NONE',  ( 33.17209381374411237, -281.3243500973783853, -239.4288554009896188 ) ) ;
#67925=CARTESIAN_POINT ( 'NONE',  ( -40.35782140593648393, -296.0944997354601469, -194.8101823289173353 ) ) ;
#67926=CARTESIAN_POINT ( 'NONE',  ( -106.6781908969197730, -284.8151411543809104, -236.8730446974805091 ) ) ;
#67927=CARTESIAN_POINT ( 'NONE',  ( 25.37985504928040470, -278.0810450631452113, -310.9268726455360934 ) ) ;
#67928=CARTESIAN_POINT ( 'NONE',  ( -78.61250283441957265, -282.4167719108331767, -331.0558570297703795 ) ) ;
#67930=CARTESIAN_POINT ( 'NONE',  ( -10.68046693611383269, -284.3995729524770013, -200.2045769020429873 ) ) ;
#67931=CARTESIAN_POINT ( 'NONE',  ( -69.79380305693813114, -275.6144242129291797, -338.8382095829550167 ) ) ;
#67932=CARTESIAN_POINT ( 'NONE',  ( 128.9467878515196162, -299.5541904835127980, -190.0176033293537898 ) ) ;
#67933=CARTESIAN_POINT ( 'NONE',  ( -6.012240014580857661, -282.1366229225249072, -336.3783140037922976 ) ) ;
#67934=CARTESIAN_POINT ( 'NONE',  ( -5.125019354807623273, -281.6719430170912801, -200.8622388538459234 ) ) ;
#67935=CARTESIAN_POINT ( 'NONE',  ( 31.21705024087159686, -286.1651879147840418, -235.8282646377669209 ) ) ;
#67936=CARTESIAN_POINT ( 'NONE',  ( 32.50368154035151491, -295.6354206608824029, -295.0013746899238072 ) ) ;
#67937=CARTESIAN_POINT ( 'NONE',  ( 24.66393884032850181, -276.5591347244908320, -226.0472569867062589 ) ) ;
#67938=CARTESIAN_POINT ( 'NONE',  ( 32.09837933787137132, -276.4523561422292914, -238.1200121733180026 ) ) ;
#67939=CARTESIAN_POINT ( 'NONE',  ( -48.60993446628410197, -277.0328083270072739, -342.5375853563188002 ) ) ;
#67940=CARTESIAN_POINT ( 'NONE',  ( -36.48184718728297327, -300.0630971103087177, -195.5274819368085275 ) ) ;
#67941=CARTESIAN_POINT ( 'NONE',  ( 10.21471392157809177, -284.7097257643019361, -212.5820914579276746 ) ) ;
#67942=CARTESIAN_POINT ( 'NONE',  ( -108.0484753211601259, -291.7879597478672622, -298.7687288566094139 ) ) ;
#67943=CARTESIAN_POINT ( 'NONE',  ( 33.95158964912825894, -292.2475451420747277, -253.2342829545661118 ) ) ;
#67945=CARTESIAN_POINT ( 'NONE',  ( -0.07651123015015320883, -292.2296127269679573, -207.5646755421059311 ) ) ;
#67947=CARTESIAN_POINT ( 'NONE',  ( 12.22654771181180422, -289.4604863441891212, -328.8801859431951584 ) ) ;
#67948=CARTESIAN_POINT ( 'NONE',  ( -69.79300284164453672, -280.2645642908326522, -204.8430110196242993 ) ) ;
#67949=CARTESIAN_POINT ( 'NONE',  ( -110.5090319631680558, -295.1820766518945902, -293.3840905849748424 ) ) ;
#67950=CARTESIAN_POINT ( 'NONE',  ( 37.61840056338752447, -287.9880703834617179, -253.1476460686504311 ) ) ;
#67951=CARTESIAN_POINT ( 'NONE',  ( -103.0298307889525802, -284.4524052199699327, -302.3701277377415977 ) ) ;
#67952=CARTESIAN_POINT ( 'NONE',  ( -71.36758396777378266, -196.0736500916017349, -360.3844923773536379 ) ) ;
#67953=CARTESIAN_POINT ( 'NONE',  ( 200.3228602561044909, 293.1909332922194835, -82.91689554719077648 ) ) ;
#67954=CARTESIAN_POINT ( 'NONE',  ( 183.8917990829111204, 260.9239217872068934, -151.0172562811493435 ) ) ;
#67955=CARTESIAN_POINT ( 'NONE',  ( -24.31086291543331512, -276.0788206443075978, -342.4043408777426407 ) ) ;
#67956=CARTESIAN_POINT ( 'NONE',  ( -100.8574957138548740, -276.9714722583235584, -307.0687015684266612 ) ) ;
#67957=CARTESIAN_POINT ( 'NONE',  ( -64.88855040576572719, -273.3687554889528428, -198.4656779917778522 ) ) ;
#67958=CARTESIAN_POINT ( 'NONE',  ( 197.7401110981591046, 281.6830570221753192, -110.4716931870877232 ) ) ;
#67959=CARTESIAN_POINT ( 'NONE',  ( -111.3546582770964619, -276.9923150778280387, -289.7873722607557170 ) ) ;
#67961=CARTESIAN_POINT ( 'NONE',  ( -90.63335162943880619, -290.3251890686217394, -320.4148713803528494 ) ) ;
#67962=CARTESIAN_POINT ( 'NONE',  ( -85.12400900874098397, -298.2141399372649175, -210.1862912023570118 ) ) ;
#67963=CARTESIAN_POINT ( 'NONE',  ( -60.13584441126318580, -298.2568854244454997, -196.8212600872328721 ) ) ;
#67964=CARTESIAN_POINT ( 'NONE',  ( -61.01115929978592334, -295.5346636623442009, -339.4708770377285418 ) ) ;
#67966=CARTESIAN_POINT ( 'NONE',  ( -7.127621448421942674, -278.5790495386513044, -339.6313273649662960 ) ) ;
#67967=CARTESIAN_POINT ( 'NONE',  ( -37.32056822534475060, -282.5595136838723533, -347.3126315705792990 ) ) ;
#67968=CARTESIAN_POINT ( 'NONE',  ( -92.95218477867335594, -278.9545911955683550, -318.1282622478202597 ) ) ;
#67969=CARTESIAN_POINT ( 'NONE',  ( 19.13921014235693008, -278.0116105886222613, -321.2124846674767582 ) ) ;
#67970=CARTESIAN_POINT ( 'NONE',  ( -109.8079439713880276, -271.2105919967353884, -256.6963271181957680 ) ) ;
#67972=CARTESIAN_POINT ( 'NONE',  ( -99.46884663712525310, -279.2485240209946369, -231.9343046221575548 ) ) ;
#67973=CARTESIAN_POINT ( 'NONE',  ( -73.87711823577588177, -274.3827969602620556, -202.7052058461952413 ) ) ;
#67974=CARTESIAN_POINT ( 'NONE',  ( -43.16159424032478853, -287.8090210531993307, -346.6462876116061693 ) ) ;
#67976=CARTESIAN_POINT ( 'NONE',  ( -94.51991033661415997, -275.2241708475329460, -221.8062666635315736 ) ) ;
#67977=CARTESIAN_POINT ( 'NONE',  ( 20.36325729342618374, -274.8091730481162358, -320.4682806281419403 ) ) ;
#67979=CARTESIAN_POINT ( 'NONE',  ( -110.2845109548321005, -289.6667531334592240, -276.6335987572646786 ) ) ;
#67980=CARTESIAN_POINT ( 'NONE',  ( -113.8033912855467804, -283.7982951701727643, -278.5417397048719295 ) ) ;
#67981=CARTESIAN_POINT ( 'NONE',  ( 21.80639121950892800, -280.4084696783950221, -314.8733706511301307 ) ) ;
#67982=CARTESIAN_POINT ( 'NONE',  ( 18.42281383825081775, -279.4483301238203694, -222.3241270821210094 ) ) ;
#67983=CARTESIAN_POINT ( 'NONE',  ( -68.12122013930522257, -283.7246268291344222, -202.5825420988205678 ) ) ;
#67984=CARTESIAN_POINT ( 'NONE',  ( -86.25476746883335011, -291.7304969609512568, -327.2838668155660002 ) ) ;
#67985=CARTESIAN_POINT ( 'NONE',  ( 26.79843078234099352, -282.2720014819543053, -234.6795525648647356 ) ) ;
#67987=CARTESIAN_POINT ( 'NONE',  ( -44.36597912735508231, -281.5393353125747353, -346.2894771678300003 ) ) ;
#67988=CARTESIAN_POINT ( 'NONE',  ( 34.77388202715069099, -295.2866542647110464, -249.7147806820009919 ) ) ;
#67989=CARTESIAN_POINT ( 'NONE',  ( -79.33189979869551678, -277.7340169711944782, -206.9671569916252736 ) ) ;
#67991=CARTESIAN_POINT ( 'NONE',  ( -30.35922307239078322, -284.9641743501890119, -345.2027737658839897 ) ) ;
#67993=CARTESIAN_POINT ( 'NONE',  ( -58.55821692027766545, -293.7000674796388466, -197.8409579521736532 ) ) ;
#67994=CARTESIAN_POINT ( 'NONE',  ( 25.65071260390737251, -274.1016340842912200, -311.1625599911782274 ) ) ;
#67995=CARTESIAN_POINT ( 'NONE',  ( 16.19402474984885387, -285.9860469761973150, -215.2422919611237830 ) ) ;
#67996=CARTESIAN_POINT ( 'NONE',  ( -84.32281430234569086, -289.7929009646389886, -213.4470131931893491 ) ) ;
#67998=CARTESIAN_POINT ( 'NONE',  ( -13.64210883320424550, -275.4229271545212328, -339.9816481934057606 ) ) ;
#67999=CARTESIAN_POINT ( 'NONE',  ( -42.49878882750282827, -293.2574717372093573, -344.4169747200843972 ) ) ;
#68001=CARTESIAN_POINT ( 'NONE',  ( 1.365254254040420667, -291.0388908463314692, -204.5399510668778760 ) ) ;
#68002=CARTESIAN_POINT ( 'NONE',  ( -101.6988352794953272, -286.6423603212411422, -234.1370966021339086 ) ) ;
#68003=CARTESIAN_POINT ( 'NONE',  ( -23.51857418612149075, -287.1177954561270553, -345.1332922237016305 ) ) ;
#68004=CARTESIAN_POINT ( 'NONE',  ( 18.20915749410774254, -288.2948384041913528, -222.0964607717205865 ) ) ;
#68006=CARTESIAN_POINT ( 'NONE',  ( 33.24040722790052627, -288.6110441941652311, -289.8045471496445771 ) ) ;
#68007=CARTESIAN_POINT ( 'NONE',  ( 32.92701375854250045, -295.8843552410523330, -297.5771913473021755 ) ) ;
#68009=CARTESIAN_POINT ( 'NONE',  ( 39.24273979168306425, -288.7360698089669881, -268.6781801777773353 ) ) ;
#68010=CARTESIAN_POINT ( 'NONE',  ( -20.47184734261383809, -274.9171282316470979, -344.0675230881357720 ) ) ;
#68011=CARTESIAN_POINT ( 'NONE',  ( -108.6352528280842620, -278.5165877008970483, -299.3951262290981390 ) ) ;
#68012=CARTESIAN_POINT ( 'NONE',  ( 15.15001990267774445, -280.4353872017491085, -213.9822642933030465 ) ) ;
#68013=CARTESIAN_POINT ( 'NONE',  ( -41.99552101784625080, -299.9730955149311171, -195.8615290241952778 ) ) ;
#68015=CARTESIAN_POINT ( 'NONE',  ( -16.59483519063446622, -284.3199027427820056, -198.2334636998320150 ) ) ;
#68017=CARTESIAN_POINT ( 'NONE',  ( -107.4382629279140815, -276.3702192487625098, -294.9576466081902595 ) ) ;
#68019=CARTESIAN_POINT ( 'NONE',  ( 23.47030784637063050, -280.1498402592361572, -314.2793817525225677 ) ) ;
#68022=CARTESIAN_POINT ( 'NONE',  ( -41.36740103434616600, -275.5818269897894766, -346.5746112612732190 ) ) ;
#68023=CARTESIAN_POINT ( 'NONE',  ( -96.95801376481071543, -297.4714418944759018, -313.7024241678608973 ) ) ;
#68024=CARTESIAN_POINT ( 'NONE',  ( -16.24014190140286118, -281.7060405804369907, -344.1468828225698644 ) ) ;
#68025=CARTESIAN_POINT ( 'NONE',  ( -68.15742442424215142, -298.5785342241073295, -203.9109760038682566 ) ) ;
#68026=CARTESIAN_POINT ( 'NONE',  ( -48.91205145469294280, -299.2230245407114353, -194.6809123958559269 ) ) ;
#68027=CARTESIAN_POINT ( 'NONE',  ( -65.81747857712534255, -273.3357858488736838, -203.1211185138928386 ) ) ;
#68028=CARTESIAN_POINT ( 'NONE',  ( 32.45594189482856251, -295.9111951901935527, -297.9494606870847520 ) ) ;
#68029=CARTESIAN_POINT ( 'NONE',  ( 39.09083458752916584, -287.8408934426537940, -280.1210784354585712 ) ) ;
#68030=CARTESIAN_POINT ( 'NONE',  ( -107.1723533280117664, -277.0058302471460365, -241.4994813475094304 ) ) ;
#68031=CARTESIAN_POINT ( 'NONE',  ( -75.66552285833041935, -289.3822901575002788, -337.1464802698899348 ) ) ;
#68032=CARTESIAN_POINT ( 'NONE',  ( 5.974172654105434077, -287.5073803721600143, -329.4763519531848601 ) ) ;
#68033=CARTESIAN_POINT ( 'NONE',  ( -33.61265125226293549, -290.0989374305921160, -195.4538763760898235 ) ) ;
#68035=CARTESIAN_POINT ( 'NONE',  ( -114.4693872376281121, -273.8646567567205921, -270.3778293100139649 ) ) ;
#68036=CARTESIAN_POINT ( 'NONE',  ( 10.15051113916259773, -287.8843490789424777, -325.9480786204479728 ) ) ;
#68038=CARTESIAN_POINT ( 'NONE',  ( -113.9726313964366398, -285.4262601498192566, -275.7133541240098111 ) ) ;
#68039=CARTESIAN_POINT ( 'NONE',  ( 27.85886593504272213, -292.0781285254188901, -229.7426767115387634 ) ) ;
#68040=CARTESIAN_POINT ( 'NONE',  ( 33.57236284135233007, -282.7933954745735150, -242.3310736313474365 ) ) ;
#68041=CARTESIAN_POINT ( 'NONE',  ( -28.30001377769427862, -281.4796305174583040, -194.3371446734178107 ) ) ;
#68042=CARTESIAN_POINT ( 'NONE',  ( -88.89579363589730576, -283.6343667361678058, -322.1154870453477201 ) ) ;
#68043=CARTESIAN_POINT ( 'NONE',  ( -110.3457092059037734, -296.2438530954198086, -294.8440642628838191 ) ) ;
#68044=CARTESIAN_POINT ( 'NONE',  ( -76.84330527862451277, -274.8261163084321765, -208.3863919401575515 ) ) ;
#68045=CARTESIAN_POINT ( 'NONE',  ( 21.49459017924854720, -290.9388526922273286, -224.4041811176136605 ) ) ;
#68046=CARTESIAN_POINT ( 'NONE',  ( -38.07099108983459956, -272.8377349151577391, -196.9676670429302874 ) ) ;
#68049=CARTESIAN_POINT ( 'NONE',  ( -76.87149117972481349, -285.5057223933551427, -333.4990821760551967 ) ) ;
#68050=CARTESIAN_POINT ( 'NONE',  ( 21.14088101435581990, -295.3032293000255777, -319.9724091729534621 ) ) ;
#68051=CARTESIAN_POINT ( 'NONE',  ( -105.3056440876494264, -284.8422927826481441, -297.4208877177229624 ) ) ;
#68052=CARTESIAN_POINT ( 'NONE',  ( -20.19037303947784778, -275.8958727986864687, -345.2398092751535614 ) ) ;
#68053=CARTESIAN_POINT ( 'NONE',  ( -4.655015081991387582, -293.1229551579453982, -200.7558494476321869 ) ) ;
#68054=CARTESIAN_POINT ( 'NONE',  ( 38.46619441944143603, -285.7069203248997837, -271.5558411501484102 ) ) ;
#68056=CARTESIAN_POINT ( 'NONE',  ( 13.26138474120823929, -293.0707595175329061, -212.3518765364509306 ) ) ;
#68057=CARTESIAN_POINT ( 'NONE',  ( -100.3200380702444647, -290.3769257703779658, -307.4176524460082192 ) ) ;
#68060=CARTESIAN_POINT ( 'NONE',  ( 199.1258471188012891, 285.7378598522153084, -96.31343096893938593 ) ) ;
#68062=CARTESIAN_POINT ( 'NONE',  ( -105.1589923710728129, -285.6160149279586449, -305.4552379626754828 ) ) ;
#68063=CARTESIAN_POINT ( 'NONE',  ( -55.56934967048407970, -277.3380690714490129, -190.3538533559490702 ) ) ;
#68065=CARTESIAN_POINT ( 'NONE',  ( -104.4015821500162389, -283.0755834202888082, -299.9786515715932751 ) ) ;
#68066=CARTESIAN_POINT ( 'NONE',  ( -113.2790060983146390, -278.0609958136691944, -282.9813340477207930 ) ) ;
#68067=CARTESIAN_POINT ( 'NONE',  ( -86.71234504026892864, -281.3639507542870319, -214.1244053769936500 ) ) ;
#68068=CARTESIAN_POINT ( 'NONE',  ( 181.7509201127585641, 251.9238600837264812, -165.7362594150378072 ) ) ;
#68069=CARTESIAN_POINT ( 'NONE',  ( 0.5601939280280614497, -281.1320317273629712, -336.7241987376779093 ) ) ;
#68070=CARTESIAN_POINT ( 'NONE',  ( -22.09988701013485368, -284.2683207579281088, -197.2359498752210527 ) ) ;
#68071=CARTESIAN_POINT ( 'NONE',  ( -92.29287814772024490, -275.1371476508344358, -218.1821028393644895 ) ) ;
#68072=CARTESIAN_POINT ( 'NONE',  ( -66.07156677837504333, -295.9309451761309333, -337.5368814992067996 ) ) ;
#68074=CARTESIAN_POINT ( 'NONE',  ( 36.13426802308160291, -292.2784513809542091, -273.5268045503592589 ) ) ;
#68075=CARTESIAN_POINT ( 'NONE',  ( -112.6920800975441210, -279.0105158767562443, -285.7765014058771271 ) ) ;
#68076=CARTESIAN_POINT ( 'NONE',  ( -21.93402851751446292, -274.2551363543284424, -199.0056440822282298 ) ) ;
#68077=CARTESIAN_POINT ( 'NONE',  ( 34.43729592382244675, -274.1294622653417719, -243.3561511257005918 ) ) ;
#68079=CARTESIAN_POINT ( 'NONE',  ( -9.249494481875080609, -272.4190927161547506, -200.7666451320033332 ) ) ;
#68080=CARTESIAN_POINT ( 'NONE',  ( -6.022488948093698724, -296.0737774010196972, -340.0584156749062004 ) ) ;
#68083=CARTESIAN_POINT ( 'NONE',  ( -76.27970941358364598, -284.6653751929001146, -332.5344097842944393 ) ) ;
#68084=CARTESIAN_POINT ( 'NONE',  ( -112.8939062428196252, -286.2094609425076897, -278.4751899405060271 ) ) ;
#68085=CARTESIAN_POINT ( 'NONE',  ( -97.62110101696028153, -283.3248167661758998, -311.8049650682105494 ) ) ;
#68086=CARTESIAN_POINT ( 'NONE',  ( 18.02203024092520423, -274.6415159115558140, -319.1787189590065736 ) ) ;
#68087=CARTESIAN_POINT ( 'NONE',  ( 29.26971607245713258, -283.8505789622883526, -303.2465046600732421 ) ) ;
#68088=CARTESIAN_POINT ( 'NONE',  ( -71.99719536520285601, -275.9989487384877975, -335.4115308088791494 ) ) ;
#68089=CARTESIAN_POINT ( 'NONE',  ( 22.52535353554809205, -276.0434627677731214, -228.0290874512854487 ) ) ;
#68091=CARTESIAN_POINT ( 'NONE',  ( -25.43072538397962035, -281.0031068117947370, -194.4513854001695279 ) ) ;
#68092=CARTESIAN_POINT ( 'NONE',  ( -1.169915738527468330, -281.0113986848400600, -202.4558242459682162 ) ) ;
#68096=CARTESIAN_POINT ( 'NONE',  ( -5.317921177660586807, -288.3294705759100793, -201.6968400351543096 ) ) ;
#68097=CARTESIAN_POINT ( 'NONE',  ( -66.12606293550669534, -294.6359747032634573, -337.6222671332523078 ) ) ;
#68098=CARTESIAN_POINT ( 'NONE',  ( -111.1320119292167732, -290.1725358431882569, -248.7208159749096126 ) ) ;
#68099=CARTESIAN_POINT ( 'NONE',  ( 35.27405704044780776, -285.9791160856950114, -284.7417650910822431 ) ) ;
#68100=CARTESIAN_POINT ( 'NONE',  ( 35.33833199506874934, -286.2788330938241756, -281.9733345030993519 ) ) ;
#68101=CARTESIAN_POINT ( 'NONE',  ( -101.9981422329643408, -289.2790634579071138, -234.2348233834122198 ) ) ;
#68102=CARTESIAN_POINT ( 'NONE',  ( -4.430195664870769434, -287.7010193353468139, -204.7565192107494738 ) ) ;
#68103=CARTESIAN_POINT ( 'NONE',  ( -111.3304271840530646, -276.3943856895510294, -282.6358448095689369 ) ) ;
#68104=CARTESIAN_POINT ( 'NONE',  ( -3.435204156061415492, -287.0119727073325748, -338.6162696419744407 ) ) ;
#68105=CARTESIAN_POINT ( 'NONE',  ( -1.936776624305429628, -288.5212814234006942, -204.2438581886043210 ) ) ;
#68106=CARTESIAN_POINT ( 'NONE',  ( 27.31350747876188834, -286.0636770670988085, -308.6982090815802167 ) ) ;
#68107=CARTESIAN_POINT ( 'NONE',  ( 19.54236240378520861, -283.1441324987565054, -316.5069319659992289 ) ) ;
#68108=CARTESIAN_POINT ( 'NONE',  ( -48.56938332891684951, -291.1948055548065213, -344.7371740285177566 ) ) ;
#68111=CARTESIAN_POINT ( 'NONE',  ( -112.6870074786758096, -298.5531716504414703, -264.0161821276322485 ) ) ;
#68112=CARTESIAN_POINT ( 'NONE',  ( 13.24747034815653635, -280.3445444988888084, -325.7302111383315264 ) ) ;
#68113=CARTESIAN_POINT ( 'NONE',  ( -42.03386674233713194, -291.1915918114947885, -193.6659917156558777 ) ) ;
#68114=CARTESIAN_POINT ( 'NONE',  ( -104.4375144098692232, -295.3634876448812179, -239.5039730179465209 ) ) ;
#68115=CARTESIAN_POINT ( 'NONE',  ( 17.44152136826783561, -279.5408207855496698, -221.3708932315629738 ) ) ;
#68116=CARTESIAN_POINT ( 'NONE',  ( -66.35222538564052286, -271.7491693495936715, -201.8067335575473180 ) ) ;
#68117=CARTESIAN_POINT ( 'NONE',  ( -100.5823470951192320, -297.3551008953662631, -307.9027602475997583 ) ) ;
#68119=CARTESIAN_POINT ( 'NONE',  ( -37.23494835315388229, -296.5333528485438137, -194.0537167287832858 ) ) ;
#68120=CARTESIAN_POINT ( 'NONE',  ( 21.48768313162443988, -292.4464461992631072, -318.4760026626552758 ) ) ;
#68121=CARTESIAN_POINT ( 'NONE',  ( -3.380336603583590449, -293.9350932193924564, -205.0771175991985444 ) ) ;
#68124=CARTESIAN_POINT ( 'NONE',  ( 34.10528807209895064, -294.1469700896925019, -254.5574449005835049 ) ) ;
#68127=CARTESIAN_POINT ( 'NONE',  ( -22.08418670521753313, -280.8777261988713008, -344.1555289087579581 ) ) ;
#68128=CARTESIAN_POINT ( 'NONE',  ( -73.30240448022638589, -295.5433849891717841, -333.8892829371502557 ) ) ;
#68129=CARTESIAN_POINT ( 'NONE',  ( 6.925008835452445943, -282.4682459897093736, -333.4299571026047602 ) ) ;
#68130=CARTESIAN_POINT ( 'NONE',  ( -6.834608772088241579, -282.3695609618431490, -201.2194681513061028 ) ) ;
#68132=CARTESIAN_POINT ( 'NONE',  ( -4.779032676873494978, -286.1361284858115823, -200.6085769527804530 ) ) ;
#68133=CARTESIAN_POINT ( 'NONE',  ( -66.00622989085336201, -289.6760666325096167, -201.2214890212815419 ) ) ;
#68136=CARTESIAN_POINT ( 'NONE',  ( -4.480114855683805963, -281.1068724959789620, -339.2436382176995266 ) ) ;
#68137=CARTESIAN_POINT ( 'NONE',  ( -38.92762112559048404, -287.9919465014788216, -347.0356076482782441 ) ) ;
#68139=CARTESIAN_POINT ( 'NONE',  ( -42.42470478329951078, -296.7174574360030306, -343.9858657197873413 ) ) ;
#68140=CARTESIAN_POINT ( 'NONE',  ( -5.513536827198955770, -278.0668759923802895, -339.8274718220787349 ) ) ;
#68141=CARTESIAN_POINT ( 'NONE',  ( 37.85882738418492721, -291.6435903541458288, -275.9429713176689916 ) ) ;
#68142=CARTESIAN_POINT ( 'NONE',  ( -104.4598356075898806, -278.6051343877720683, -241.5992790906739742 ) ) ;
#68143=CARTESIAN_POINT ( 'NONE',  ( -11.15524869941154229, -292.5507348674066179, -197.8946551662417335 ) ) ;
#68144=CARTESIAN_POINT ( 'NONE',  ( -112.4746515569167542, -282.5297587967270374, -278.3832004006295620 ) ) ;
#68146=CARTESIAN_POINT ( 'NONE',  ( -81.35156202801275072, -279.6507961037555674, -331.0911163483391988 ) ) ;
#68147=CARTESIAN_POINT ( 'NONE',  ( -42.41796037625191929, -294.1764873077721063, -343.4202723044344907 ) ) ;
#68148=CARTESIAN_POINT ( 'NONE',  ( -107.4472716918866126, -270.9055020910105895, -243.1027146468452429 ) ) ;
#68151=CARTESIAN_POINT ( 'NONE',  ( -35.65547483204182555, -294.5381148762191970, -343.4157022015315306 ) ) ;
#68153=CARTESIAN_POINT ( 'NONE',  ( -82.13390479932374433, -287.1952119285918457, -326.4764044574609443 ) ) ;
#68154=CARTESIAN_POINT ( 'NONE',  ( -78.06745106268971313, -296.5775661449000040, -205.2901304115516439 ) ) ;
#68155=CARTESIAN_POINT ( 'NONE',  ( 2.470005846205419964, -287.8892437244465441, -205.0286885176707017 ) ) ;
#68156=CARTESIAN_POINT ( 'NONE',  ( 23.50832415670129194, -287.9453286307909252, -310.7110436777061295 ) ) ;
#68157=CARTESIAN_POINT ( 'NONE',  ( -110.8585195312119254, -279.9966025379366101, -276.1524647362191445 ) ) ;
#68158=CARTESIAN_POINT ( 'NONE',  ( -99.30808309524991273, -298.8665981674900536, -229.7943730339071919 ) ) ;
#68159=CARTESIAN_POINT ( 'NONE',  ( -71.11077110766973419, -278.3910264473072402, -205.1796293333489984 ) ) ;
#68160=ORIENTED_EDGE ( 'NONE', *, *, #75186, .F. ) ;
#68161=CARTESIAN_POINT ( 'NONE',  ( -73.26697940214680216, -297.2561194965205686, -202.2205851647523502 ) ) ;
#68162=CARTESIAN_POINT ( 'NONE',  ( -19.75521800301713071, -294.2000285052232584, -197.9750500273278817 ) ) ;
#68163=CARTESIAN_POINT ( 'NONE',  ( 35.92924609118153256, -294.8866867874316426, -249.3897366780731488 ) ) ;
#68165=CARTESIAN_POINT ( 'NONE',  ( -104.1374862354397948, -290.8027716561011289, -300.1882116075222484 ) ) ;
#68167=CARTESIAN_POINT ( 'NONE',  ( -16.93614702093297097, -290.4525111718118637, -197.3959284710996371 ) ) ;
#68168=CARTESIAN_POINT ( 'NONE',  ( -71.67118871967464599, -297.2520938694800634, -205.8986914482326256 ) ) ;
#68171=CARTESIAN_POINT ( 'NONE',  ( -111.9660414447004513, -292.2741067489715761, -254.3646712383266220 ) ) ;
#68172=CARTESIAN_POINT ( 'NONE',  ( 25.18497378105907814, -295.4090924074130839, -220.4570493818173702 ) ) ;
#68173=CARTESIAN_POINT ( 'NONE',  ( -35.92363991557247260, -288.0701400896182349, -195.5412173182348283 ) ) ;
#68174=CARTESIAN_POINT ( 'NONE',  ( -10.81714863463806786, -272.3985159329216117, -200.3308781809405161 ) ) ;
#68175=CARTESIAN_POINT ( 'NONE',  ( 5.995614212063472337, -276.5648012480422722, -209.7731193528359768 ) ) ;
#68176=CARTESIAN_POINT ( 'NONE',  ( -65.85638376163679197, -289.7560601331077805, -201.5852350712984560 ) ) ;
#68177=CARTESIAN_POINT ( 'NONE',  ( -92.41950375270855034, -279.6898567445617232, -322.4627236557338392 ) ) ;
#68180=CARTESIAN_POINT ( 'NONE',  ( -4.789213084710878476, -281.9602129049083032, -335.8151343286834276 ) ) ;
#68181=CARTESIAN_POINT ( 'NONE',  ( -101.8295820842718200, -279.0839187408105886, -311.9646886768086915 ) ) ;
#68183=CARTESIAN_POINT ( 'NONE',  ( 39.01713346955680350, -280.2702631687407120, -264.2506966091918912 ) ) ;
#68184=CARTESIAN_POINT ( 'NONE',  ( -23.25451841258840702, -108.0230548315861228, -359.5793218185942237 ) ) ;
#68185=CARTESIAN_POINT ( 'NONE',  ( 34.98333684742553373, -276.8208671833418180, -296.2454659780066777 ) ) ;
#68187=CARTESIAN_POINT ( 'NONE',  ( -18.73791950962220909, -275.8074798397020118, -196.3024849677360066 ) ) ;
#68188=CARTESIAN_POINT ( 'NONE',  ( -85.28047601435908120, -298.1948066931273615, -330.5268031993605859 ) ) ;
#68193=CARTESIAN_POINT ( 'NONE',  ( -58.76639227940843568, -290.4154094221062223, -340.5226909414288343 ) ) ;
#68194=CARTESIAN_POINT ( 'NONE',  ( -43.08307500583523364, -290.8838399972848947, -346.1305750769485030 ) ) ;
#68195=CARTESIAN_POINT ( 'NONE',  ( -110.4390666189930243, -289.8899706868205044, -271.1782348167046734 ) ) ;
#68196=CARTESIAN_POINT ( 'NONE',  ( -71.03362207790604543, -285.1270369143106791, -201.1918957886914541 ) ) ;
#68198=CARTESIAN_POINT ( 'NONE',  ( 28.85978928636847485, -280.3905914401466362, -303.0930240330241645 ) ) ;
#68199=CARTESIAN_POINT ( 'NONE',  ( 34.90863849092423976, -289.6337747367565498, -287.4126297407460697 ) ) ;
#68200=CARTESIAN_POINT ( 'NONE',  ( -69.32744702836673412, -281.9607209728453654, -336.7649611624587465 ) ) ;
#68201=CARTESIAN_POINT ( 'NONE',  ( -24.80864878983320665, -281.5305769905262423, -197.9445031696770343 ) ) ;
#68202=CARTESIAN_POINT ( 'NONE',  ( 37.59787051185729467, -288.7028931890693002, -287.0609102581877323 ) ) ;
#68203=CARTESIAN_POINT ( 'NONE',  ( -107.2878432503601687, -279.3237200250767387, -249.2536429075893523 ) ) ;
#68205=CARTESIAN_POINT ( 'NONE',  ( -82.63030655195812813, -288.4508128464818242, -332.1425945407843301 ) ) ;
#68206=CARTESIAN_POINT ( 'NONE',  ( -113.9915834790967040, -285.4313054464715265, -264.2712388212321457 ) ) ;
#68207=CARTESIAN_POINT ( 'NONE',  ( -29.47546774090680088, -286.6416090093147204, -193.8258366333480751 ) ) ;
#68208=CARTESIAN_POINT ( 'NONE',  ( -106.1730206436254349, -284.3934411963727484, -294.8272514909809843 ) ) ;
#68211=CARTESIAN_POINT ( 'NONE',  ( 25.45561829809514620, -294.8438349271464745, -227.8801642848519577 ) ) ;
#68212=CARTESIAN_POINT ( 'NONE',  ( 6.318747573993888977, -293.1580178845388787, -333.2513205825137561 ) ) ;
#68213=CARTESIAN_POINT ( 'NONE',  ( 30.49145158158179925, -274.9811050137151938, -298.1016518714695280 ) ) ;
#68214=CARTESIAN_POINT ( 'NONE',  ( -27.76876061533236495, -294.2823461513569896, -346.7142190754476019 ) ) ;
#68215=CARTESIAN_POINT ( 'NONE',  ( -108.4155023662685693, -289.2868959687370989, -250.8874848063960599 ) ) ;
#68216=CARTESIAN_POINT ( 'NONE',  ( -15.31229921200150201, -293.0030087938605448, -341.0739173088455232 ) ) ;
#68217=CARTESIAN_POINT ( 'NONE',  ( -37.56648963734183866, -293.2543901205146426, -196.9518768416542116 ) ) ;
#68219=CARTESIAN_POINT ( 'NONE',  ( 37.77384621546699606, -291.5874995121845359, -273.1329623433663869 ) ) ;
#68220=CARTESIAN_POINT ( 'NONE',  ( -87.40220017547704856, -297.7500733112210014, -326.2773113011045893 ) ) ;
#68221=CARTESIAN_POINT ( 'NONE',  ( 28.44436102823925694, -288.9279034904681112, -302.5418980369116753 ) ) ;
#68222=CARTESIAN_POINT ( 'NONE',  ( -2.211680179745054708, -278.5693669085690658, -337.0266150843143578 ) ) ;
#68223=CARTESIAN_POINT ( 'NONE',  ( -108.2944544808214857, -276.9784784927340411, -299.2352477078088668 ) ) ;
#68224=CARTESIAN_POINT ( 'NONE',  ( -44.02561982015154030, -273.3184745797630057, -193.7008442194582472 ) ) ;
#68225=CARTESIAN_POINT ( 'NONE',  ( 3.514360123374058897, -278.6856735298910053, -208.0730814171312488 ) ) ;
#68226=CARTESIAN_POINT ( 'NONE',  ( -28.71208679880496462, -275.3444723414158375, -346.1239116492341168 ) ) ;
#68228=CARTESIAN_POINT ( 'NONE',  ( -84.80930274944560665, -294.4071799903408078, -326.5356153282622245 ) ) ;
#68229=CARTESIAN_POINT ( 'NONE',  ( 145.2857639756989272, -299.5541904835127980, -195.3611179825600175 ) ) ;
#68230=CARTESIAN_POINT ( 'NONE',  ( -40.53522992484867160, -298.8138391489502510, -197.2567971679214622 ) ) ;
#68232=CARTESIAN_POINT ( 'NONE',  ( -59.56674070809860666, -287.3586909929717308, -342.3642732730834837 ) ) ;
#68233=CARTESIAN_POINT ( 'NONE',  ( -1.720774803308078083, -274.3715100236110516, -206.6275005022664857 ) ) ;
#68234=CARTESIAN_POINT ( 'NONE',  ( 23.28745962536372005, -288.1868200511356122, -317.8492315087341353 ) ) ;
#68236=CARTESIAN_POINT ( 'NONE',  ( -91.86041495851810623, -275.2768696531442743, -218.5954614916149126 ) ) ;
#68237=CARTESIAN_POINT ( 'NONE',  ( -100.2889047179441349, -294.0045845158685438, -310.9243262591206758 ) ) ;
#68238=CARTESIAN_POINT ( 'NONE',  ( -76.68402382037567122, -282.7614468443223359, -336.4253907082803039 ) ) ;
#68240=CARTESIAN_POINT ( 'NONE',  ( -106.7874521163989243, -276.9229081003919646, -241.9013258546824261 ) ) ;
#68242=CARTESIAN_POINT ( 'NONE',  ( -69.17601360528942678, -290.4187796333781080, -204.2132330037402994 ) ) ;
#68245=CARTESIAN_POINT ( 'NONE',  ( -34.76370661218703617, -290.0843910714747267, -195.4054337353889252 ) ) ;
#68246=CARTESIAN_POINT ( 'NONE',  ( -40.82692550182953539, -275.5277826960543166, -196.7000708261558373 ) ) ;
#68247=CARTESIAN_POINT ( 'NONE',  ( 36.62601983310198506, -283.2191621828485495, -289.5283477820594840 ) ) ;
#68248=CARTESIAN_POINT ( 'NONE',  ( -79.67961082692174557, -295.5035787369413924, -207.9613405089926346 ) ) ;
#68249=CARTESIAN_POINT ( 'NONE',  ( -33.49622495927432198, -283.0024352086145427, -343.2723347003428671 ) ) ;
#68250=CARTESIAN_POINT ( 'NONE',  ( -32.67162431688959146, -275.5374047398941570, -196.9075937844483235 ) ) ;
#68251=CARTESIAN_POINT ( 'NONE',  ( -35.39625786534305263, -274.8799912201071152, -197.2129780881582519 ) ) ;
#68252=EDGE_CURVE ( 'NONE', #46969, #44141, #12179, .T. ) ;
#68253=CARTESIAN_POINT ( 'NONE',  ( -24.84118108081210607, -284.8929889110902423, -344.3647450824703924 ) ) ;
#68255=CARTESIAN_POINT ( 'NONE',  ( 203.2380858836131097, 291.9636489450776367, -53.99999999997883293 ) ) ;
#68256=CARTESIAN_POINT ( 'NONE',  ( 8.904463510063092002, -294.2704878251129799, -331.9264682474528740 ) ) ;
#68260=CARTESIAN_POINT ( 'NONE',  ( 36.57525178469694538, -285.4809262143061801, -305.9938812882205070 ) ) ;
#68261=CARTESIAN_POINT ( 'NONE',  ( -113.0756011663440006, -277.9120231582376164, -257.3790128287753873 ) ) ;
#68262=CARTESIAN_POINT ( 'NONE',  ( -71.79216514076699696, -290.0044462979988680, -202.3789893732148073 ) ) ;
#68263=CARTESIAN_POINT ( 'NONE',  ( -109.8788954254723507, -286.2431167119542579, -257.2876007725129739 ) ) ;
#68264=CARTESIAN_POINT ( 'NONE',  ( -64.68696564924297832, -279.1741722590903692, -339.1920628701112719 ) ) ;
#68265=CARTESIAN_POINT ( 'NONE',  ( -30.95136032721581643, -287.5566518426239782, -194.2048369856267129 ) ) ;
#68266=CARTESIAN_POINT ( 'NONE',  ( 29.95665205232298334, -283.9903010137520027, -303.5839280930067048 ) ) ;
#68267=CARTESIAN_POINT ( 'NONE',  ( -1.465847451629220144, -276.7564478725773256, -338.4927787524290466 ) ) ;
#68268=CARTESIAN_POINT ( 'NONE',  ( -108.6572321136195569, -278.0167069861469145, -299.3972145195943426 ) ) ;
#68269=CARTESIAN_POINT ( 'NONE',  ( -109.5781508691519690, -298.7055692796266158, -252.3308367490608077 ) ) ;
#68272=CARTESIAN_POINT ( 'NONE',  ( -30.59740699726062019, -296.2753177241256139, -194.5984209097469204 ) ) ;
#68274=CARTESIAN_POINT ( 'NONE',  ( -103.1891897845255386, -277.6304879278584963, -302.1341105276584358 ) ) ;
#68275=CARTESIAN_POINT ( 'NONE',  ( -64.77230194073887048, -274.9068642136576841, -198.8237855755641590 ) ) ;
#68276=CARTESIAN_POINT ( 'NONE',  ( 37.31671867858363356, -280.8355964471062407, -288.2760612169074079 ) ) ;
#68277=CARTESIAN_POINT ( 'NONE',  ( -27.72680229456249634, -287.9360790159931298, -196.9749629409670035 ) ) ;
#68278=CARTESIAN_POINT ( 'NONE',  ( -69.22046592836221635, -296.9840475676032270, -339.7039994193829671 ) ) ;
#68279=CARTESIAN_POINT ( 'NONE',  ( -99.67640017537755170, -297.1633500057298534, -314.9745205380372681 ) ) ;
#68280=CARTESIAN_POINT ( 'NONE',  ( -4.039535456207898889, -294.4924206869389423, -203.3319647022740924 ) ) ;
#68281=CARTESIAN_POINT ( 'NONE',  ( -27.28745629830472907, -278.1799192287834330, -196.1537974063413401 ) ) ;
#68282=CARTESIAN_POINT ( 'NONE',  ( 31.34089874792687880, -283.0946764400395068, -241.6554598822298772 ) ) ;
#68283=CARTESIAN_POINT ( 'NONE',  ( -110.7425282997226077, -270.7508960706601897, -256.5143776799616262 ) ) ;
#68284=CARTESIAN_POINT ( 'NONE',  ( -78.70816290299524098, -285.1996186883256996, -334.3553065605329380 ) ) ;
#68285=CARTESIAN_POINT ( 'NONE',  ( 34.58477660331920589, -286.6594758771205420, -284.5966240585956371 ) ) ;
#68286=CARTESIAN_POINT ( 'NONE',  ( 30.98277457338434004, -281.3561911198370353, -305.6467941564162629 ) ) ;
#68287=CARTESIAN_POINT ( 'NONE',  ( -11.11022278200930558, -92.70253263746865002, -359.4537332136167151 ) ) ;
#68289=CARTESIAN_POINT ( 'NONE',  ( -27.82959668005257470, -285.8429938832449011, -197.9621720322206500 ) ) ;
#68291=CARTESIAN_POINT ( 'NONE',  ( -109.0091602172492742, -285.2831866890015249, -297.8086170479778616 ) ) ;
#68292=CARTESIAN_POINT ( 'NONE',  ( 35.39887449299214950, -275.7938246196474097, -263.4145137880428820 ) ) ;
#68293=CARTESIAN_POINT ( 'NONE',  ( 2.547410411992344415, -285.3694003799847110, -204.9633536586277103 ) ) ;
#68294=CARTESIAN_POINT ( 'NONE',  ( -86.30506999379602462, -290.3115942056789436, -211.2660713682429332 ) ) ;
#68295=CARTESIAN_POINT ( 'NONE',  ( 31.80429870901055978, -282.0629695675908692, -236.8974348519450075 ) ) ;
#68297=CARTESIAN_POINT ( 'NONE',  ( -50.83620284106032017, -281.4028644689976204, -195.2571490623167278 ) ) ;
#68298=CARTESIAN_POINT ( 'NONE',  ( 37.17240806842435319, -282.1273476364965518, -289.6844709857626867 ) ) ;
#68299=CARTESIAN_POINT ( 'NONE',  ( -53.35057174420112602, -280.7666405000205145, -340.3538533559490702 ) ) ;
#68300=CARTESIAN_POINT ( 'NONE',  ( -89.44128332668068992, -230.9695510001336061, -347.9586317399256927 ) ) ;
#68302=CARTESIAN_POINT ( 'NONE',  ( 36.52081155437959126, -277.7109644354906663, -282.6897660608909746 ) ) ;
#68303=CARTESIAN_POINT ( 'NONE',  ( 202.4137727338654145, 295.8836245966012939, -68.61462046017487637 ) ) ;
#68304=CARTESIAN_POINT ( 'NONE',  ( 35.24378545467292412, -279.7976016100379866, -287.8278912963958760 ) ) ;
#68305=CARTESIAN_POINT ( 'NONE',  ( -84.13372638231025746, -296.7377939835836855, -214.1309973625218959 ) ) ;
#68306=CARTESIAN_POINT ( 'NONE',  ( -8.528442555772940636, -291.9269967620080024, -199.0216261750705939 ) ) ;
#68308=CARTESIAN_POINT ( 'NONE',  ( -111.9585833985336905, -271.4497082950938989, -253.4608515288946364 ) ) ;
#68309=CARTESIAN_POINT ( 'NONE',  ( 17.49860077288287741, -285.2524054886260387, -220.9561968347129550 ) ) ;
#68310=CARTESIAN_POINT ( 'NONE',  ( 31.97340496418030042, -295.0635297477839458, -243.7851573310300068 ) ) ;
#68311=CARTESIAN_POINT ( 'NONE',  ( -27.78892319592413074, -287.4911834976902583, -197.4914539913472709 ) ) ;
#68313=CARTESIAN_POINT ( 'NONE',  ( -7.293385877938820983, -293.3779557772207909, -199.7074822970287471 ) ) ;
#68314=CARTESIAN_POINT ( 'NONE',  ( -86.96604037179409374, -284.2574985429677668, -324.0532075999353765 ) ) ;
#68315=CARTESIAN_POINT ( 'NONE',  ( 98.32702654663349051, -298.5100415232777209, -193.7851615946195523 ) ) ;
#68316=CARTESIAN_POINT ( 'NONE',  ( -103.6538913608810901, -290.8474934253744664, -309.2845285084534339 ) ) ;
#68317=CARTESIAN_POINT ( 'NONE',  ( -39.21648186493953148, -292.5215923412303596, -193.4324765471042724 ) ) ;
#68318=CARTESIAN_POINT ( 'NONE',  ( -97.34769812036847725, -290.1393520099832699, -311.9556679138568143 ) ) ;
#68319=ORIENTED_EDGE ( 'NONE', *, *, #88201, .F. ) ;
#68321=CARTESIAN_POINT ( 'NONE',  ( -97.27173917898515754, -299.0416701196417080, -223.9861427894485928 ) ) ;
#68322=CARTESIAN_POINT ( 'NONE',  ( -31.27612358005698567, -272.9220556158824138, -193.9854961107881763 ) ) ;
#68324=CARTESIAN_POINT ( 'NONE',  ( 35.26769376072147111, -280.4802999492753202, -260.4293321346249854 ) ) ;
#68327=CARTESIAN_POINT ( 'NONE',  ( 1.170053370301559426, -274.0596261781940939, -203.7397505483738200 ) ) ;
#68328=CARTESIAN_POINT ( 'NONE',  ( -50.05467972473267224, -296.3668478065745262, -197.7726347324097844 ) ) ;
#68329=CARTESIAN_POINT ( 'NONE',  ( -46.02953020763133196, -279.0237719941371779, -344.1376773496667738 ) ) ;
#68330=CARTESIAN_POINT ( 'NONE',  ( 35.33540859630638664, -273.4946662308361738, -255.1694151051649442 ) ) ;
#68332=CARTESIAN_POINT ( 'NONE',  ( -70.66144693004908106, -298.8076802801734857, -204.9489263732471045 ) ) ;
#68333=CARTESIAN_POINT ( 'NONE',  ( -110.5496402674577752, -297.5812541623145080, -274.2112573753506695 ) ) ;
#68334=CARTESIAN_POINT ( 'NONE',  ( -113.4336187099429338, -298.0897629919161318, -275.3079574863053267 ) ) ;
#68335=CARTESIAN_POINT ( 'NONE',  ( -41.08527851115144358, -272.0255016400885211, -195.0478156383719579 ) ) ;
#68336=CARTESIAN_POINT ( 'NONE',  ( 32.85037379755767262, -294.4738350036436714, -290.8258589516847223 ) ) ;
#68337=CARTESIAN_POINT ( 'NONE',  ( 31.38511609544448433, -291.7783707396216641, -244.0552317994517750 ) ) ;
#68339=CARTESIAN_POINT ( 'NONE',  ( 38.43040694093095055, -275.8765122366463629, -256.9399099676472247 ) ) ;
#68340=CARTESIAN_POINT ( 'NONE',  ( -63.30870623302911326, -273.8708978526993860, -202.1221554521191592 ) ) ;
#68341=CARTESIAN_POINT ( 'NONE',  ( -83.59844996041638865, -282.3562785599247036, -331.3670858172334306 ) ) ;
#68343=CARTESIAN_POINT ( 'NONE',  ( -109.0853113604347300, -283.9379855821192109, -256.0273824345195521 ) ) ;
#68344=CARTESIAN_POINT ( 'NONE',  ( -91.13980850780355070, -281.8143853667122585, -322.8567555219859742 ) ) ;
#68346=CARTESIAN_POINT ( 'NONE',  ( 19.62630006753686374, -274.7814137089202973, -316.9644618080894247 ) ) ;
#68347=CARTESIAN_POINT ( 'NONE',  ( -10.45842673334823303, -282.4029203368400545, -200.2900439322175430 ) ) ;
#68349=CARTESIAN_POINT ( 'NONE',  ( -55.12692399563955092, -272.2269772601271711, -196.2657319900211519 ) ) ;
#68350=CARTESIAN_POINT ( 'NONE',  ( -109.6693238589066510, -280.2895844533979357, -290.8243355635115108 ) ) ;
#68352=CARTESIAN_POINT ( 'NONE',  ( -104.1701412615792037, -286.9375009851185041, -234.9889348342551898 ) ) ;
#68354=CARTESIAN_POINT ( 'NONE',  ( -73.78304147019487402, -287.5357767546639138, -335.9273842735322546 ) ) ;
#68356=CARTESIAN_POINT ( 'NONE',  ( -93.03574360256133957, -296.0241336871748672, -222.5369376958423402 ) ) ;
#68357=CARTESIAN_POINT ( 'NONE',  ( -31.80243948563547107, -287.1212288633412300, -344.4408493656098926 ) ) ;
#68358=CARTESIAN_POINT ( 'NONE',  ( -35.93751134800100289, -122.5594593288581251, -363.2174194532766478 ) ) ;
#68359=CARTESIAN_POINT ( 'NONE',  ( -111.0053523957496537, -294.7338470623768103, -256.1979106822892049 ) ) ;
#68360=CARTESIAN_POINT ( 'NONE',  ( -106.0463765469124695, -283.4619170499775009, -237.1590820651039735 ) ) ;
#68361=CARTESIAN_POINT ( 'NONE',  ( -5.228600245311270989, -282.0821595823695134, -203.9142276586865989 ) ) ;
#68362=CARTESIAN_POINT ( 'NONE',  ( 1.555906525634688453, -280.7795316778975234, -335.6370722843251428 ) ) ;
#68363=CARTESIAN_POINT ( 'NONE',  ( -92.41172517849986434, -289.8682286249937761, -318.3563034840150863 ) ) ;
#68364=CARTESIAN_POINT ( 'NONE',  ( 24.63642525851434684, -283.5229760691759111, -310.1295930600817314 ) ) ;
#68365=CARTESIAN_POINT ( 'NONE',  ( -33.47749448940577821, -283.8051381041314585, -343.4330752799006632 ) ) ;
#68367=CARTESIAN_POINT ( 'NONE',  ( 19.03897906200381840, -288.8392426917267812, -220.2878646290233746 ) ) ;
#68368=CARTESIAN_POINT ( 'NONE',  ( -31.91166361358936143, -298.2850575700418290, -193.3609690682164057 ) ) ;
#68370=CARTESIAN_POINT ( 'NONE',  ( -71.40280104847005305, -273.6147269303191933, -201.3043195910106249 ) ) ;
#68371=CARTESIAN_POINT ( 'NONE',  ( -2.899238311503552712, -294.4896234450193333, -204.1375298169641326 ) ) ;
#68373=CARTESIAN_POINT ( 'NONE',  ( -37.37352853689063892, -288.5519495502701943, -195.3611179825600175 ) ) ;
#68375=CARTESIAN_POINT ( 'NONE',  ( 37.31354789722783494, -273.6697087536383606, -279.5496824014452386 ) ) ;
#68377=CARTESIAN_POINT ( 'NONE',  ( -113.5090896857543470, -294.9976274434279730, -266.7526290622055853 ) ) ;
#68378=CARTESIAN_POINT ( 'NONE',  ( -1.665644115893663457, -273.8868551248680205, -206.5415199493936882 ) ) ;
#68379=CARTESIAN_POINT ( 'NONE',  ( -79.94718285793359769, -292.9845490272139727, -210.1696928222670522 ) ) ;
#68380=CARTESIAN_POINT ( 'NONE',  ( -61.84940986627871240, -285.1351080055624720, -340.2530856550145018 ) ) ;
#68381=CARTESIAN_POINT ( 'NONE',  ( -112.5500953213806810, -291.8063263903147799, -283.9369107372662597 ) ) ;
#68382=CARTESIAN_POINT ( 'NONE',  ( -102.8026306123124840, -292.3886370004836976, -230.6588780488229986 ) ) ;
#68383=CARTESIAN_POINT ( 'NONE',  ( -34.30331926453491320, -294.8462094232859840, -343.2978593839272889 ) ) ;
#68384=CARTESIAN_POINT ( 'NONE',  ( 30.61158399337896441, -289.1351492818308770, -238.6223117233984397 ) ) ;
#68385=CARTESIAN_POINT ( 'NONE',  ( 23.74600930128720222, -281.0933142952720800, -223.4643003413286522 ) ) ;
#68386=CARTESIAN_POINT ( 'NONE',  ( -100.4395098995483835, -294.0739341297344254, -312.0247741560880286 ) ) ;
#68387=CARTESIAN_POINT ( 'NONE',  ( -10.70402646358210497, -282.5476109601004850, -342.6634163795613404 ) ) ;
#68388=CARTESIAN_POINT ( 'NONE',  ( -5.553785854370113739, -278.6118679223745289, -337.9131540086680729 ) ) ;
#68390=CARTESIAN_POINT ( 'NONE',  ( -35.76141371055521034, -275.1721490433179724, -346.1223526039944431 ) ) ;
#68391=DIRECTION ( 'NONE',  ( -1.000000000000000000, -0.000000000000000000, -0.000000000000000000 ) ) ;
#68393=CARTESIAN_POINT ( 'NONE',  ( -3.598530781493743280, -282.1018834281535987, -335.1778115412341776 ) ) ;
#68395=CARTESIAN_POINT ( 'NONE',  ( -69.80812268687949995, -280.8391996572095763, -200.9642382458584109 ) ) ;
#68396=CARTESIAN_POINT ( 'NONE',  ( 34.63777792396833632, -286.2725735048651359, -243.6820072050919066 ) ) ;
#68397=CARTESIAN_POINT ( 'NONE',  ( 27.10605077755610282, -294.8197083538659058, -233.8633771306119797 ) ) ;
#68398=CARTESIAN_POINT ( 'NONE',  ( 23.73873534974671173, -277.7646669189965678, -315.9200997434085707 ) ) ;
#68400=CARTESIAN_POINT ( 'NONE',  ( 30.11620404028058218, -277.3380741327698615, -306.5663667808615855 ) ) ;
#68401=CARTESIAN_POINT ( 'NONE',  ( -83.00841149244826056, -277.5303596797073737, -327.3783635016786207 ) ) ;
#68402=CARTESIAN_POINT ( 'NONE',  ( -85.26803842849682269, -299.3889410165205049, -212.8208872898309778 ) ) ;
#68403=CARTESIAN_POINT ( 'NONE',  ( 8.058917278216032543, -284.6737996454291419, -210.8077113090986359 ) ) ;
#68405=CARTESIAN_POINT ( 'NONE',  ( 23.15242131724019004, -293.8558825388064975, -317.9869452891306878 ) ) ;
#68406=CARTESIAN_POINT ( 'NONE',  ( -67.71606923919844689, -291.0442730697384945, -340.2455806194385559 ) ) ;
#68407=CARTESIAN_POINT ( 'NONE',  ( -9.597799629979137492, -291.3435645212375675, -202.4506187485807800 ) ) ;
#68409=CARTESIAN_POINT ( 'NONE',  ( -70.62453610134701876, -290.1965488427768491, -201.5798768970310277 ) ) ;
#68410=CARTESIAN_POINT ( 'NONE',  ( 18.49549683846597503, -292.5505262355009677, -223.3048227419540410 ) ) ;
#68412=CARTESIAN_POINT ( 'NONE',  ( -74.26637465608381206, -290.6108195064770143, -337.5926324791993238 ) ) ;
#68413=CARTESIAN_POINT ( 'NONE',  ( -102.2502051271011112, -279.6615629961774516, -236.6238740934600173 ) ) ;
#68414=CARTESIAN_POINT ( 'NONE',  ( -65.41599023963952675, -296.6140840750867937, -198.9368152003324042 ) ) ;
#68415=CARTESIAN_POINT ( 'NONE',  ( -3.541653042610806601, -287.1379948536681468, -201.2751283789181684 ) ) ;
#68416=CARTESIAN_POINT ( 'NONE',  ( 36.66971422386825452, -287.6178714900088949, -249.0045766847676134 ) ) ;
#68417=CARTESIAN_POINT ( 'NONE',  ( -107.0047570717433416, -284.5953885792574738, -292.2505214474406330 ) ) ;
#68418=CARTESIAN_POINT ( 'NONE',  ( -56.60324186021520632, -169.1846951020332028, -364.3055494911789083 ) ) ;
#68419=CARTESIAN_POINT ( 'NONE',  ( -49.43407259941375997, -154.1845681105646690, -363.5609398828140115 ) ) ;
#68420=CARTESIAN_POINT ( 'NONE',  ( 64.45001422827949966, 46.57074262894973771, -315.3000494332260359 ) ) ;
#68421=CARTESIAN_POINT ( 'NONE',  ( -95.40740334110685694, -277.1245358482831875, -314.8692727168392480 ) ) ;
#68422=CARTESIAN_POINT ( 'NONE',  ( 13.93776827101168614, -275.2326265235146252, -322.8211349177072975 ) ) ;
#68423=CARTESIAN_POINT ( 'NONE',  ( -46.11662604878426919, -297.4513314995372752, -193.9246896369507738 ) ) ;
#68424=CARTESIAN_POINT ( 'NONE',  ( 26.83260473079646502, -24.62933982865472871, -342.1012798676335933 ) ) ;
#68425=CARTESIAN_POINT ( 'NONE',  ( -86.78931057167142171, -276.4077431730805756, -328.8105140398925528 ) ) ;
#68426=CARTESIAN_POINT ( 'NONE',  ( -64.96754881973922124, -275.4464210113846434, -201.6831460444351762 ) ) ;
#68427=CARTESIAN_POINT ( 'NONE',  ( -84.72017325600741344, -290.2179862707740767, -326.0450523073967588 ) ) ;
#68428=CARTESIAN_POINT ( 'NONE',  ( 53.34045889417781439, -299.9632562302277847, -193.5105485799727489 ) ) ;
#68429=CARTESIAN_POINT ( 'NONE',  ( -101.5018370342409355, -297.6037442819738317, -227.8753335946865093 ) ) ;
#68430=CARTESIAN_POINT ( 'NONE',  ( -4.334760257134855799, -294.7712040644221361, -335.4868812224659109 ) ) ;
#68432=CARTESIAN_POINT ( 'NONE',  ( -74.60437101017137707, -279.4641283677482306, -336.0939678938331099 ) ) ;
#68433=CARTESIAN_POINT ( 'NONE',  ( -35.90663495134732841, -282.5422953164523960, -347.2993016609133292 ) ) ;
#68434=CARTESIAN_POINT ( 'NONE',  ( -66.88662933562555679, -278.3903727189822348, -337.3723529123301432 ) ) ;
#68435=CARTESIAN_POINT ( 'NONE',  ( 35.91476065463498912, -277.5690847940529693, -290.5954492241596654 ) ) ;
#68436=CARTESIAN_POINT ( 'NONE',  ( -36.45646440760401674, -296.6381726008356168, -196.7721045031088067 ) ) ;
#68438=CARTESIAN_POINT ( 'NONE',  ( -74.01144054981590159, -277.7207229415566303, -333.4826685173074452 ) ) ;
#68439=CARTESIAN_POINT ( 'NONE',  ( -64.85183790945018245, -274.5046859558662504, -198.6019186033956885 ) ) ;
#68440=CARTESIAN_POINT ( 'NONE',  ( -7.130177354123384603, -287.3488695339653418, -340.6643978980135330 ) ) ;
#68441=CARTESIAN_POINT ( 'NONE',  ( -35.59653940537977945, -276.0741778120893173, -195.3686308519964143 ) ) ;
#68442=CARTESIAN_POINT ( 'NONE',  ( 3.173569438467552573, -275.0943706692889918, -335.2085705235602973 ) ) ;
#68444=CARTESIAN_POINT ( 'NONE',  ( -13.24431162253579686, -287.9281277036228062, -339.4401856805684474 ) ) ;
#68445=CARTESIAN_POINT ( 'NONE',  ( -111.7783908071708083, -283.6582752681582633, -289.7133926939125672 ) ) ;
#68446=CARTESIAN_POINT ( 'NONE',  ( 35.47847237912510820, -279.9651470506128703, -283.6681983543881529 ) ) ;
#68447=CARTESIAN_POINT ( 'NONE',  ( 31.62885886734168750, -279.7856446449549708, -244.5548020066396475 ) ) ;
#68448=CARTESIAN_POINT ( 'NONE',  ( -111.6643547565761878, -282.6968924718063363, -265.3442634026137625 ) ) ;
#68449=CARTESIAN_POINT ( 'NONE',  ( 21.13005604134814419, -290.1987140432833030, -317.3498309153775381 ) ) ;
#68450=CARTESIAN_POINT ( 'NONE',  ( -105.8906099957172131, -280.1073635266718043, -243.9855501237966848 ) ) ;
#68453=CARTESIAN_POINT ( 'NONE',  ( 30.02419410728393601, -279.4860640992655476, -234.6356978869577574 ) ) ;
#68454=CARTESIAN_POINT ( 'NONE',  ( 18.86257163776771861, -294.8616755083610315, -220.6820767023252188 ) ) ;
#68455=CARTESIAN_POINT ( 'NONE',  ( -88.23590778428064141, -277.5907254898050951, -213.9363571171152216 ) ) ;
#68457=CARTESIAN_POINT ( 'NONE',  ( -1.412905491629123267, -277.2140329782872641, -334.0816913708131324 ) ) ;
#68458=CARTESIAN_POINT ( 'NONE',  ( -95.73174578151045466, -285.9016969049153545, -317.7166410043448082 ) ) ;
#68459=DIRECTION ( 'NONE',  ( 0.000000000000000000, 0.000000000000000000, -1.000000000000000000 ) ) ;
#68460=CARTESIAN_POINT ( 'NONE',  ( -86.43000992025280027, -291.6472956920073898, -327.8724194175006801 ) ) ;
#68462=CARTESIAN_POINT ( 'NONE',  ( 0.2138159796696542936, -285.7362339578068031, -203.3107220206265424 ) ) ;
#68463=CARTESIAN_POINT ( 'NONE',  ( -47.08007906786437502, -290.3262565216114126, -197.2064572312184225 ) ) ;
#68465=CARTESIAN_POINT ( 'NONE',  ( 31.71946125282903850, -274.5713978015491534, -295.6445288702159928 ) ) ;
#68466=CARTESIAN_POINT ( 'NONE',  ( 8.980753267418275954, -292.5487825161296200, -328.4366111618166428 ) ) ;
#68469=CARTESIAN_POINT ( 'NONE',  ( -11.37085642590842305, -290.8642047948958975, -198.5544600203934920 ) ) ;
#68470=CARTESIAN_POINT ( 'NONE',  ( -111.1176266111509960, -286.1087937281242830, -273.6943695669645535 ) ) ;
#68471=CARTESIAN_POINT ( 'NONE',  ( -67.67029256810022275, -287.6845465779465485, -340.0328518220001115 ) ) ;
#68472=CARTESIAN_POINT ( 'NONE',  ( -5.560483446708854416, -287.9037906763186356, -203.9745701137698575 ) ) ;
#68473=DIRECTION ( 'NONE',  ( 0.9951408606192332362, 0.000000000000000000, -0.09846150276129254919 ) ) ;
#68474=CARTESIAN_POINT ( 'NONE',  ( 33.86511549150084477, -288.1331623484406919, -253.5084609292994742 ) ) ;
#68475=CARTESIAN_POINT ( 'NONE',  ( 36.74489105905452391, -295.7088925685389427, -284.1999065763107524 ) ) ;
#68476=CARTESIAN_POINT ( 'NONE',  ( -112.3401198887111150, -276.5095152970703793, -279.9716269123249504 ) ) ;
#68477=CARTESIAN_POINT ( 'NONE',  ( -22.93869317498068483, -277.2061377411561693, -346.0347151488948043 ) ) ;
#68478=CARTESIAN_POINT ( 'NONE',  ( -33.58601733639245168, -290.1789309195158353, -194.8945091649860615 ) ) ;
#68479=CARTESIAN_POINT ( 'NONE',  ( -114.2108522076812278, -278.6082686985297414, -265.8740857157554274 ) ) ;
#68480=CARTESIAN_POINT ( 'NONE',  ( -47.52146415016976277, -299.9021612129894834, -196.3613431997065391 ) ) ;
#68482=CARTESIAN_POINT ( 'NONE',  ( -112.0911152258861279, -282.4733336966953630, -276.4869313375109527 ) ) ;
#68484=CARTESIAN_POINT ( 'NONE',  ( -96.26770673127754208, -276.0671235951129461, -315.5118790952369636 ) ) ;
#68485=CARTESIAN_POINT ( 'NONE',  ( 35.90659070774783856, -279.7596681712798841, -286.5351921248577014 ) ) ;
#68487=CARTESIAN_POINT ( 'NONE',  ( -25.89326948699024200, -275.3887493745876327, -345.8040844350275052 ) ) ;
#68488=CARTESIAN_POINT ( 'NONE',  ( -103.1602145007605742, -298.5192524226204682, -237.1018371702075456 ) ) ;
#68490=CARTESIAN_POINT ( 'NONE',  ( 4.366011256174946453, -281.4245215264569424, -334.7819320839103625 ) ) ;
#68491=CARTESIAN_POINT ( 'NONE',  ( -108.1941796040006949, -297.2489620859068395, -288.9399586035870584 ) ) ;
#68492=CARTESIAN_POINT ( 'NONE',  ( -103.4322961883367071, -298.3732025329255748, -231.7166789724855960 ) ) ;
#68493=CARTESIAN_POINT ( 'NONE',  ( -64.57273150917869486, -273.3533365635586279, -202.5939748196624350 ) ) ;
#68494=CARTESIAN_POINT ( 'NONE',  ( 27.96384264065048697, -295.0596889621393188, -233.3744308843161264 ) ) ;
#68495=CARTESIAN_POINT ( 'NONE',  ( 38.02306859478124323, -287.5206255436393690, -254.5127466676893562 ) ) ;
#68496=CARTESIAN_POINT ( 'NONE',  ( 29.44289890549298505, -274.1629952905269079, -306.2506345709406332 ) ) ;
#68497=CARTESIAN_POINT ( 'NONE',  ( 14.60214286555750007, -288.1784971513300206, -327.2738228997328065 ) ) ;
#68499=CARTESIAN_POINT ( 'NONE',  ( 27.87310784581042356, -286.1582819267348441, -236.9260460160904813 ) ) ;
#68500=CARTESIAN_POINT ( 'NONE',  ( -104.2091343531707395, -289.0023027498201600, -236.2798331643919880 ) ) ;
#68502=CARTESIAN_POINT ( 'NONE',  ( 125.5584997210034572, 149.0310057319917405, -265.9501514013184078 ) ) ;
#68503=CARTESIAN_POINT ( 'NONE',  ( 17.86791605282812156, -287.7418860257988626, -318.2896183447253406 ) ) ;
#68505=CARTESIAN_POINT ( 'NONE',  ( -70.35802020846388416, -284.4179180454589186, -339.6773586285799524 ) ) ;
#68506=CARTESIAN_POINT ( 'NONE',  ( -36.36927160204471221, -291.1228179276945980, -193.5895777901128554 ) ) ;
#68507=CARTESIAN_POINT ( 'NONE',  ( 37.64203410756061174, -283.3245629837664410, -283.9939352902941891 ) ) ;
#68508=CARTESIAN_POINT ( 'NONE',  ( 14.81283117316611353, -282.0835769441939078, -214.3136896195209715 ) ) ;
#68509=CARTESIAN_POINT ( 'NONE',  ( -101.7722262708617507, -283.9165226295036177, -304.7864499276090555 ) ) ;
#68510=CARTESIAN_POINT ( 'NONE',  ( -73.79233343604141737, -279.5362303213421455, -335.9224547970185313 ) ) ;
#68511=CARTESIAN_POINT ( 'NONE',  ( -113.9432200410501963, -296.4543085083787446, -278.1846176485049682 ) ) ;
#68512=CARTESIAN_POINT ( 'NONE',  ( -98.26130087192044016, -274.4359593214324491, -229.1601332729453873 ) ) ;
#68513=CARTESIAN_POINT ( 'NONE',  ( 23.95265296160118496, -290.9913533261548650, -227.7375408787310960 ) ) ;
#68514=CARTESIAN_POINT ( 'NONE',  ( -33.77949833879921471, -297.0181016681536903, -197.0526761339389168 ) ) ;
#68517=CARTESIAN_POINT ( 'NONE',  ( -109.1437777325013911, -286.2172707393778524, -290.0503612655991219 ) ) ;
#68518=CIRCLE ( 'NONE', #468, 0.5000000000000004441 ) ;
#68519=CARTESIAN_POINT ( 'NONE',  ( -8.491511416715544769, -295.7630534574070111, -341.4748132229282191 ) ) ;
#68520=CARTESIAN_POINT ( 'NONE',  ( -110.4203193355407677, -285.1602312421156853, -273.6509839895760479 ) ) ;
#68521=CARTESIAN_POINT ( 'NONE',  ( 36.65559886206544604, -274.8681280489462324, -290.8360653234958022 ) ) ;
#68522=CARTESIAN_POINT ( 'NONE',  ( 22.12514995342863600, -293.5479771148287682, -221.6065640571553104 ) ) ;
#68523=CARTESIAN_POINT ( 'NONE',  ( -10.41050100170151538, -284.5392949572897123, -199.4884431808527268 ) ) ;
#68524=CARTESIAN_POINT ( 'NONE',  ( 30.87821778903895265, -293.4239062900076647, -234.5842530023379311 ) ) ;
#68526=CARTESIAN_POINT ( 'NONE',  ( -45.36055653205941951, -289.4898311840251495, -342.9406290633068011 ) ) ;
#68529=CARTESIAN_POINT ( 'NONE',  ( 161.0643044244293947, 217.6531385774068781, -202.3978598018051400 ) ) ;
#68530=CARTESIAN_POINT ( 'NONE',  ( -101.9419003248663387, -286.6089114077928457, -229.7468115569240865 ) ) ;
#68531=CARTESIAN_POINT ( 'NONE',  ( -85.28047601435909542, -294.9094976428776818, -210.1954327657594206 ) ) ;
#68533=CARTESIAN_POINT ( 'NONE',  ( 34.87395367371294697, -280.3067725856217862, -257.7466255189837625 ) ) ;
#68534=CARTESIAN_POINT ( 'NONE',  ( -110.6478376737737648, -277.9214608828444852, -294.0264843838895104 ) ) ;
#68535=CARTESIAN_POINT ( 'NONE',  ( -16.43329065755524354, -282.3231646729834097, -198.5080259311049247 ) ) ;
#68536=CARTESIAN_POINT ( 'NONE',  ( 198.7516057561506955, 282.3040474041899301, -110.9336064257162349 ) ) ;
#68537=CARTESIAN_POINT ( 'NONE',  ( 22.05370066387754235, -280.7766784376967735, -318.4524602079354167 ) ) ;
#68538=CARTESIAN_POINT ( 'NONE',  ( -16.69322455083104373, -284.3401677694872660, -198.5750222909682918 ) ) ;
#68539=CARTESIAN_POINT ( 'NONE',  ( -105.7384823260575359, -274.8371672387395961, -237.7699280267998176 ) ) ;
#68540=B_SPLINE_SURFACE_WITH_KNOTS ( 'NONE', 3, 3, ( 
 ( #14917, #2100, #23414, #30507, #74055, #67442, #8268, #52280, #30051, #37148, #38052, #66055, #58932, #66961, #30991, #31448, #38539, #88718, #2569, #22469, #22023, #60337, #72673, #36678, #65600, #713, #29598, #87321, #75459, #82081, #10580, #47018, #24806, #68837, #26195, #55089, #69291, #82559, #40374, #4420, #76866, #18165, #25267, #33774, #11046, #39916, #89174, #53692, #90561, #3487, #18630, #47496, #38984, #24326, #76405, #89636, #68359, #60798, #83958, #17707, #61729, #32839, #83474, #39443, #46560, #19107, #53203, #32380, #46101, #11527, #54603, #17239, #3965, #62196, #54144, #75006, #10118, #90115, #61281, #91026, #47962, #67897, #3020, #83013, #11991, #31906, #25719, #33298, #40840, #69759, #4890, #71647, #13418, #6305, #19562, #49839, #93397, #5385, #27614, #27140, #13879, #64095, #91520, #70250, #84414, #35173, #50308, #7233, #41798, #34250, #71176, #63156, #6780, #92935, #79213, #35657, #34712, #42263, #20972, #26676, #56511, #42732, #92451, #20520, #57440, #77810, #28096, #63626, #85370, #56025, #64572, #56983, #55566, #28549, #85821, #49388, #78736, #14356, #84880, #78280, #70709, #20031, #86281, #12959, #48908, #21434, #43216, #72117, #62687, #48428, #77332, #91987, #12466, #41313, #5840, #81499, #65484, #16646, #30395, #37936, #22359, #29009, #51233, #87669, #601, #15730, #66845, #1980, #16190, #29484, #81047, #45042, #23754, #58824, #65949, #74402, #22819, #51688, #36108, #58369, #37483, #44120, #59287, #88133, #79671, #65026, #23291, #36569, #15260, #7684, #30871, #87211, #8607, #73495, #52164, #80121, #73024, #59765, #126, #8152, #86750, #73943, #1509, #57894, #80577, #9058, #1060, #21912, #50786, #37035, #29939, #88606, #66393, #52617, #45500, #44591, #14812, #43667, #72562, #68245, #54489, #39327, #61162, #4308, #24688, #39796, #10461, #75346, #67780, #11411, #75804, #38417, #83357, #46903, #3369, #32729, #54964, #2906, #32257, #82446, #60684, #89999, #53571, #31790, #68718, #90449, #18993, #33186, #82895, #62076, #10002, #9532, #25154, #90909, #83840, #38873, #47846, #3848, #40262, #89524, #2458, #17594, #54028, #46444, #18051, #69179, #26075, #18507, #10928, #47371, #76285, #67326, #61617, #25606, #31334, #60221, #89060, #24210, #53085, #81964, #17120, #45986, #74891, #26559, #76748, #63980, #77216, #55913, #48315, #42619, #12344, #49272, #20402, #71061, #27024, #70131, #6671, #40727, #91870, #33654, #6193, #42143, #69644, #27494, #49731, #41681, #21325, #11876, #77694, #41193, #78628, #71538, #4772, #62563, #48786, #78167, #34136, #12843, #85715, #56392, #13305, #91404, #92820, #13770, #19449, #70599, #5267, #27983, #35060, #55448, #84299, #63039, #56874, #64461, #84765, #19915, #5726, #85254, #34601, #20860, #63511, #35548, #28439, #92339, #93288, #57332, #86174, #86512, #14119, #57211, #29245, #79894, #8385, #87440, #72337, #22586, #93170, #92693, #93623, #51461, #44362, #28322, #73272, #86986, #835, #78968, #85597, #42983, #50551, #86052, #7456, #29717, #58599, #72789, #21201, #43892, #7913, #80350, #21675, #28781, #37264, #79448, #14584, #27863, #50073, #358, #7010, #22139, #51007, #42500, #56755, #15033, #71889, #35882, #64344, #15491, #64799, #65253, #36338, #36803, #57666, #43441, #20744, #49615, #58140, #78510, #65724, #13648, #71413, #6545, #35423, #31111, #10702, #66170, #67094, #30633, #68015, #32026, #87899, #30168, #38179, #38656, #23532, #2227, #75125, #16888, #9781, #23051, #53329, #3144, #8837, #59998, #59533, #17369, #67560, #1286, #73725, #51929, #2689, #53809, #59051, #45276, #37715, #74657, #66621, #10235, #31570, #82677, #39103, #88837, #45745, #24450, #80819, #23987, #46221, #52860, #81738, #60923, #81278, #60460, #89295, #82215, #88382, #89770, #24932, #15968, #17826, #46679, #16424, #75582, #44822, #1745, #52401, #74179, #9297, #39560, #47140, #83133, #25383, #18284, #68482, #61402, #54263, #76050, #90234, #3618, #32505, #93266, #65356, #22236, #44463, #29812, #14686, #58693, #35527, #35041, #35979, #87537, #80445, #64440, #15590, #29352, #36908, #21304, #27963, #50177, #86614, #28420, #43541, #65826, #933, #15130, #57311, #79993, #43993, #22684, #57768, #64899, #73368, #21784, #50660, #63955, #86153, #36441, #43086, #58244, #87087, #78605, #92795, #51107, #79073, #14225, #6647, #51557, #71990, #7556, #72438, #72890, #7108, #93715, #56852, #85693, #28880, #20839, #8014, #463, #49710, #79546, #13750, #42598, #71513, #8480, #9398, #66719, #10333, #68112, #30263, #66266, #74275, #74757, #59636, #38282, #17465, #52959, #45851, #59155, #89393, #39200, #44919, #67195, #1847, #53431, #9876, #37359, #16065, #87999, #38752, #89870, #46773, #81372, #73821, #16986, #8934, #46315, #67656, #25031, #75219, #2331, #81836, #60555, #1381, #31210, #82315, #60095, #88934, #3238, #24083, #2782, #30734, #32128, #61024, #16521, #53902, #31663, #23152, #52036, #24547, #82770, #17922, #80922, #37812, #88483, #23630, #52495, #45372, #83700, #12702, #61494, #76149, #75674, #41542, #41057, #62904, #5123, #69052, #77553, #11282, #76619, #3719, #47237, #25941, #69983, #39661, #40136, #70466, #91740, #63374, #4181, #33055, #54822, #92204, #33515, #61944, #5594, #34468, #19317, #18862, #84169, #32605, #68583, #90326, #20259, #25480, #54359, #10799, #26892, #91262, #11742, #55779, #84632, #83233, #19781, #85109, #55319, #18380, #27360, #90781, #47719, #77080, #48652, #40595, #69509, #4640, #48179, #56249, #12211, #34000, #62421, #26426, #65704, #49595, #78491, #57645, #34926, #50053, #49135, #28302, #64779, #21182, #78949, #29227, #86493, #13629, #21656, #85578, #816, #57192, #72317, #35862, #22121, #35402, #92673, #7895, #50532, #78032, #14099, #43873, #42480, #63841, #13172, #71393, #42963, #58122, #58580, #71868, #79430, #93604, #43422, #29696, #15014, #6990, #28762, #72770, #36784, #79874, #42007, #86033, #87419, #27843, #6526, #70923, #6054, #14566, #36320, #7438, #64322, #50989, #93148, #65234, #56732, #20725, #340, #86967, #80329, #23030, #82192, #9760, #10212, #80800, #51909, #66600, #39080, #74157, #87878, #46197, #75102, #59977, #1722, #31089, #44343, #15472, #73253, #60899, #8365, #37246, #22567, #38635, #38156, #52379, #67538, #31546, #66149, #2667, #32002, #2205, #59031, #67994, #44803, #1266, #23964, #60438, #30148, #51441, #15948, #88816, #89274, #52838, #81714, #16864, #16401, #3122, #73704, #8813, #45723, #37694, #23510, #30609, #59511, #67071, #88360, #81256, #24424, #74633, #45252, #53307, #9273, #17346, #5374, #20510, #77801, #64086, #77323, #40829, #49830, #63617, #24908, #56014, #85812, #91510, #11981, #55078, #26666, #91978, #6295, #6771, #63147, #34704, #12951, #85361, #71639, #56974, #27131, #41789, #20963, #78727, #84871, #70700, #55556, #92925, #35164, #70241, #28087, #5831, #47952, #83947, #92442, #20021, #13870, #27605, #49378, #19099, #56502, #78271, #13410, #41304, #84404, #42722, #76855, #12456, #69749, #42253, #71167, #4880, #35646, #89748, #48899, #33764, #62676, #19553, #34241, #66384, #30384, #86272, #28540, #36559, #37026, #21903, #592, #73485, #15251, #8143, #21424, #51678, #1500, #7224, #29474, #28999, #15721, #65940, #93387, #72107, #50298, #1051, #52155, #9049, #43658, #36098, #73014 ),
 ( #80567, #57431, #79204, #14347, #29930, #44582, #58815, #44111, #87658, #58362, #81037, #65018, #118, #22809, #43206, #65474, #64563, #72553, #80112, #87202, #22350, #8597, #37474, #57885, #59277, #86741, #16181, #7675, #88123, #51222, #23281, #50776, #79662, #45033, #73933, #14802, #2898, #32722, #38408, #52608, #1970, #67317, #38865, #46895, #47362, #9992, #75337, #53563, #32248, #18498, #3840, #67771, #82435, #61607, #90441, #31781, #17585, #59756, #76277, #88596, #30862, #37927, #25144, #46434, #60675, #54020, #75796, #23745, #82887, #66833, #10453, #74392, #83350, #60212, #81490, #39319, #18043, #16637, #45491, #9520, #68237, #10919, #3358, #61155, #89990, #89513, #54481, #2447, #31325, #39787, #89051, #24678, #24200, #17111, #68710, #25598, #53077, #81954, #45975, #74882, #77686, #47838, #27977, #19442, #34595, #91864, #78161, #91397, #54955, #63971, #12837, #40255, #70123, #6187, #11867, #26066, #69171, #40718, #12337, #20395, #20854, #77207, #48780, #27018, #5720, #85709, #71055, #41183, #55907, #35054, #92812, #5260, #84759, #69636, #13299, #49266, #84292, #42137, #19907, #62067, #4298, #41675, #34129, #56867, #70593, #63504, #33178, #92333, #49725, #90901, #48308, #11403, #83832, #4764, #18986, #76740, #27488, #56382, #85248, #33645, #62555, #26552, #63033, #55440, #50190, #28894, #44009, #42613, #79090, #44481, #65842, #66284, #43100, #14242, #57783, #1397, #36455, #72005, #8496, #37374, #22253, #86630, #87103, #6664, #71530, #7124, #79559, #35540, #35994, #21799, #72907, #64455, #64913, #73386, #950, #30282, #16, #50673, #14700, #59171, #65370, #43555, #88017, #23172, #51124, #72451, #80009, #93281, #28433, #57326, #78622, #86168, #21319, #13765, #29828, #480, #7570, #58711, #87553, #29368, #22701, #58260, #15149, #8031, #36928, #51575, #80461, #15609, #39217, #16083, #80938, #66736, #24565, #68133, #53452, #31681, #17483, #45871, #68601, #52513, #81389, #60576, #37831, #52979, #52055, #31227, #67673, #24099, #81853, #32146, #89411, #16537, #82333, #88500, #3737, #60112, #75237, #38769, #25048, #38301, #1863, #10817, #46334, #44936, #17003, #46791, #45391, #30754, #73837, #74291, #74777, #61045, #61511, #9894, #10351, #2799, #3256, #32621, #17940, #89889, #53920, #75693, #39679, #82788, #90343, #9415, #8951, #59656, #88952, #23647, #67216, #2349, #83252, #70001, #19335, #56269, #41076, #77571, #47254, #5142, #85129, #18397, #33532, #20281, #11300, #25958, #25498, #49156, #84650, #12721, #48670, #18881, #27380, #41563, #47736, #78051, #54839, #26445, #76168, #90799, #69527, #19802, #40153, #83720, #13192, #70485, #42027, #76635, #11759, #4659, #70942, #77099, #40611, #6073, #34947, #62923, #62438, #34020, #69070, #4198, #33073, #63860, #61963, #91280, #54376, #5613, #91758, #55336, #34488, #63394, #84187, #92224, #48197, #26910, #12230, #55798, #81200, #73650, #60380, #46144, #22974, #87824, #8760, #31492, #75047, #89219, #38580, #24370, #52779, #75502, #88299, #23456, #67483, #44748, #59922, #58975, #38098, #74570, #31033, #88762, #39028, #2614, #52322, #53248, #1667, #10624, #67008, #82130, #45662, #31949, #45196, #37638, #17747, #17287, #51846, #23908, #53734, #16346, #66546, #80741, #74099, #81658, #67941, #68403, #16806, #10159, #9699, #3064, #39482, #24851, #60841, #89684, #82600, #3532, #15892, #30549, #9218, #2144, #41360, #11565, #63198, #76905, #83055, #90159, #12035, #26241, #92028, #48001, #84454, #54185, #40882, #27183, #25307, #40413, #56070, #18209, #32880, #32422, #84923, #91561, #19604, #55134, #47540, #90601, #62731, #48472, #41838, #20074, #69800, #48954, #61768, #61321, #33339, #77852, #13002, #25762, #70749, #26718, #34290, #18674, #47059, #76444, #83998, #54644, #4935, #75963, #11093, #12509, #83517, #77372, #70294, #39959, #19146, #62236, #68875, #33821, #55605, #4005, #69331, #5425, #4462, #91070, #57937, #49431, #5883, #86792, #6345, #78778, #71218, #65524, #35217, #72153, #43255, #166, #49880, #92977, #29526, #63668, #21013, #56557, #29045, #65067, #92491, #50350, #72602, #64610, #44160, #34753, #6822, #64144, #7724, #642, #27659, #85411, #71693, #7269, #57024, #35696, #14850, #79255, #36146, #20559, #21951, #36606, #42309, #93436, #28135, #50824, #79708, #78319, #13458, #85862, #43703, #87252, #13919, #42776, #28590, #14396, #57480, #58406, #22398, #51270, #80163, #86321, #15301, #21473, #8195, #37973, #24248, #9096, #30911, #67817, #88173, #9569, #73979, #45079, #37519, #74927, #45537, #37076, #53122, #16682, #66881, #2493, #24727, #66429, #2018, #52202, #30431, #38457, #59801, #89558, #73533, #8642, #81534, #58861, #88642, #73065, #81084, #23790, #52654, #74438, #82002, #67363, #1548, #31370, #15772, #53610, #16228, #60259, #89096, #46024, #59322, #22858, #31828, #17158, #65985, #10038, #2942, #23333, #87708, #1096, #38908, #60719, #82481, #17628, #29977, #51724, #80616, #44631, #27058, #12382, #76320, #90946, #41228, #70167, #47410, #26110, #10963, #19483, #55483, #25641, #77252, #55003, #3403, #10496, #83876, #40298, #5302, #62115, #4809, #68281, #19027, #34172, #39365, #54524, #63074, #32294, #46938, #46480, #91904, #11911, #33689, #69678, #39830, #48349, #75840, #11446, #61200, #18084, #90483, #40760, #90036, #68754, #55945, #62599, #84800, #3885, #32762, #83393, #75383, #4342, #61650, #25188, #54061, #47881, #18543, #76785, #82932, #69213, #33219, #91442, #26593, #84332, #58298, #7162, #35580, #49766, #36037, #28936, #12878, #64954, #29407, #93321, #56425, #65413, #42179, #34633, #21360, #55, #77727, #48821, #63544, #86208, #57822, #50229, #28473, #64495, #78661, #86673, #21838, #41716, #50714, #19950, #57366, #85286, #523, #71092, #92373, #79133, #79600, #70632, #5760, #27532, #14281, #14741, #43142, #72046, #43596, #13802, #36496, #20436, #49305, #72492, #78199, #20894, #13338, #92852, #7608, #85747, #42654, #6225, #35095, #64013, #28016, #56907, #71571, #6706, #16577, #73875, #60153, #73426, #36966, #45913, #59696, #22292, #52096, #81895, #87596, #8078, #51163, #22742, #88059, #2388, #2842, #59213, #30797, #8993, #81428, #67712, #53017, #23216, #37871, #17047, #74819, #80980, #66776, #51616, #88992, #31266, #66325, #24139, #1907, #44050, #80050, #88539, #16123, #9934, #23688, #45433, #15190, #52552, #38808, #72951, #1439, #31724, #65879, #80504, #87142, #988, #74333, #9457, #38343, #15652, #29870, #44522, #44974, #58754, #8536, #37415, #67256, #30324, #61092, #26490, #47776, #48246, #25087, #89931, #10859, #77148, #18437, #32186, #84232, #19382, #4237, #39722, #69112, #82375, #24612, #17525, #5196, #46375, #53499, #60615, #76678, #47295, #53961, #12278, #41122, #33117, #68646, #62006, #75275, #10394, #39259, #89453, #68174, #3295, #82828, #11803, #76212, #90384, #40654, #69573, #17981, #4702, #70054, #40195, #46833, #75735, #3780, #32663, #90841, #33579, #61550, #25539, #54420, #26002, #62488, #54887, #83766, #18922, #83291, #11341, #91328, #55380, #19848, #62971, #55848, #34069, #48719, #77622, #12771, #41613, #70535, #91805, #84701, #26957, #65970, #46008, #37505, #52640, #16214, #2479, #15755, #73046, #81986, #2001, #58390, #88156, #24231, #29961, #44142, #87234, #58847, #30417, #38440, #38894 ),
 ( #31356, #23315, #67803, #29509, #59308, #87690, #60244, #89082, #51254, #22382, #1531, #30894, #80598, #52188, #67349, #73965, #66866, #80145, #16667, #53108, #1081, #81069, #22843, #74424, #59787, #15285, #37060, #8176, #88628, #17142, #51710, #45065, #23775, #9079, #81520, #10024, #74913, #37959, #45522, #44615, #73519, #9553, #8628, #66414, #70967, #13217, #77123, #34971, #48691, #54866, #61986, #77597, #91781, #63885, #19825, #56293, #25981, #12746, #92721, #90821, #12252, #27891, #83746, #4681, #4220, #56781, #63419, #85157, #27405, #91306, #6099, #33555, #5169, #18903, #69551, #48221, #92248, #47758, #62465, #85623, #20309, #20769, #26469, #55358, #41098, #49641, #55820, #84210, #78536, #13675, #41588, #70027, #70510, #76656, #11783, #40633, #42525, #19357, #34044, #33095, #49180, #5637, #62947, #78074, #42053, #26932, #84676, #34512, #51034, #14149, #23078, #93650, #86080, #72816, #58625, #35451, #6574, #21231, #43921, #87466, #7942, #79922, #36836, #65281, #87927, #71917, #7038, #15059, #57238, #72366, #71437, #50582, #87014, #43469, #7483, #51488, #65754, #35908, #863, #43013, #51958, #79477, #29744, #58170, #44392, #57694, #50100, #30195, #22613, #64370, #36368, #66197, #64826, #78994, #93196, #28810, #386, #80376, #80849, #29275, #22166, #37290, #1313, #15517, #73300, #86537, #8412, #59085, #14612, #15997, #28348, #21706, #8864, #89324, #38683, #75610, #60487, #3172, #66650, #24479, #10734, #37742, #52887, #39590, #30660, #45303, #44849, #68513, #10264, #32056, #68045, #38209, #46707, #74208, #45775, #1776, #16451, #88865, #39134, #59562, #9326, #3649, #60950, #32539, #67123, #2258, #24014, #61432, #2718, #31141, #90264, #25413, #82244, #81767, #53358, #88411, #23562, #52430, #83163, #81305, #60028, #73752, #89801, #17399, #74686, #24963, #53839, #16917, #82705, #54292, #46248, #9809, #67588, #31598, #75152, #17856, #5531, #76080, #47171, #32989, #84565, #34401, #19712, #91674, #77483, #12145, #34862, #18793, #47651, #26827, #4117, #19255, #18315, #91191, #33934, #84106, #48113, #92139, #55714, #76553, #48583, #54753, #63775, #26359, #41473, #5051, #85039, #4573, #61880, #70858, #12626, #11212, #77017, #13109, #11676, #90711, #40069, #40525, #40990, #27294, #27774, #69912, #70404, #62841, #63308, #92604, #77966, #68987, #56181, #20189, #49069, #41946, #5990, #25871, #56668, #83630, #69443, #55249, #33447, #62350, #85970, #85517, #22513, #50932, #72712, #14957, #78882, #87363, #21120, #86428, #13565, #57128, #35800, #79816, #49534, #49988, #51384, #7834, #73189, #14030, #42891, #64713, #8308, #43362, #71804, #15413, #44281, #29160, #93540, #280, #42415, #78427, #71326, #30092, #6456, #35331, #20663, #36722, #7375, #21585, #65641, #755, #64257, #29639, #1210, #65175, #28241, #37190, #6926, #93086, #86908, #58518, #28699, #57584, #50466, #58057, #80275, #22063, #43812, #66098, #79369, #14505, #72258, #36256, #31621, #8890, #24037, #23104, #2282, #38706, #88889, #52913, #3195, #60512, #23586, #89347, #59586, #39614, #31165, #46271, #9833, #89827, #9350, #66673, #75634, #24503, #51985, #81792, #17879, #52453, #37768, #80875, #81327, #16940, #32079, #32563, #45802, #53384, #67613, #17422, #3677, #82727, #74712, #2741, #46731, #10757, #82269, #75175, #16474, #24988, #60979, #60051, #53861, #10288, #73775, #16022, #68538, #39158, #68070, #61455, #44873, #45330, #1801, #30686, #74231, #88437, #38235, #67148, #26849, #77507, #6013, #85065, #69936, #20216, #90738, #90286, #91218, #49094, #41969, #25896, #70882, #84589, #92163, #76577, #83190, #11700, #48136, #54778, #5078, #27320, #56206, #70429, #83656, #41500, #5555, #77993, #19278, #26385, #34888, #77039, #12170, #25437, #18819, #91697, #4598, #19739, #48607, #40094, #54315, #12654, #47676, #69466, #61903, #13133, #40551, #62864, #33960, #34425, #33471, #62374, #18338, #47193, #55273, #76106, #63332, #55737, #11239, #41013, #69010, #84128, #4141, #33012, #64736, #28264, #65663, #29660, #85539, #27799, #35822, #36278, #21143, #93564, #72734, #14527, #7396, #20687, #50953, #776, #6481, #28721, #57153, #14976, #65198, #92628, #71350, #49557, #301, #51404, #9594, #42916, #35359, #72277, #64280, #7854, #29181, #80296, #36741, #57606, #43382, #22083, #56692, #86449, #43832, #21607, #50489, #58540, #78906, #58078, #79390, #86930, #85993, #87385, #79836, #22532, #14053, #50013, #15435, #44301, #73210, #63799, #78452, #13588, #93109, #42440, #71830, #6949, #83897, #67840, #19048, #32783, #40319, #24752, #31392, #53634, #90057, #2966, #18108, #69234, #4363, #18567, #31851, #83413, #47433, #26133, #61223, #68304, #76806, #25210, #54083, #38481, #60740, #39855, #46503, #61671, #90503, #82025, #67385, #25664, #38931, #17652, #10061, #33241, #89581, #10985, #75862, #54545, #82504, #75406, #62136, #2515, #10522, #89119, #76342, #3906, #60282, #82953, #11468, #3426, #24270, #53145, #39389, #32321, #90967, #55028, #17183, #46046, #46960, #68777, #47904, #74951, #20913, #56447, #49325, #62624, #92874, #42671, #48371, #70650, #70191, #56925, #13358, #40781, #19503, #33712, #78219, #93338, #50245, #84819, #77273, #20457, #12402, #49782, #42199, #28489, #78679, #77748, #85309, #64032, #69699, #5778, #85763, #41737, #63566, #6725, #27079, #71113, #12899, #34652, #5324, #13819, #6243, #4828, #71588, #35112, #92392, #28036, #57382, #34192, #27552, #19968, #63096, #35597, #64512, #86225, #21375, #11932, #91463, #26614, #55505, #84354, #48843, #41250, #91924, #55966, #79151, #16137, #44538, #66340, #8551, #72506, #80995, #14756, #80064, #7177, #50730, #29423, #73441, #43159, #79614, #44989, #1454, #66791, #43610, #7626, #58313, #1921, #36981, #36511, #9007, #37886, #22761, #87157, #87611, #36052, #72060, #64970, #23703, #73, #28951, #14299, #30340, #1005, #15207, #59230, #88076, #57837, #23232, #88555, #58769, #21856, #30815, #65426, #86691, #80518, #52112, #540, #22306, #51177, #51632, #73890, #15671, #37431, #59712, #72965, #44064, #8094, #65893, #29885, #81446, #74350, #52566, #38359, #2403, #67273, #31283, #89007, #60169, #9473, #16594, #45450, #64612, #56072, #71220, #34755, #21015, #34292, #91563, #6824, #20561, #76907, #13004, #42779, #48474, #62733, #12037, #77374, #48956, #57026, #57482, #20077, #85413, #63670, #42311, #28592, #13921, #77854, #92493, #71695, #35698, #41840, #27662, #12512, #49882, #85864, #27185, #78780, #56559, #4938, #40884, #69802, #41362, #93438, #35220, #86323, #70296, #5427, #92030, #48003, #5885, #19606, #33823, #26720, #49433, #84925, #78321, #55607, #84456, #63200, #70751, #13460, #6347, #64146, #92979, #28137, #51271, #8643, #30433, #14398, #37520, #30913, #1097, #57940, #66883, #43705, #36148, #22859, #66430, #79257, #50353, #65069, #87709, #1550, #51725, #29978, #80618, #15302, #37975, #21953, #50826, #58862, #7271, #22399, #21475, #643, #37077, #87253, #80164, #59324, #15773, #79710, #44632, #86794, #2021, #29527, #73534, #8196, #88176, #7726, #168, #73981, #23335, #43257, #44161, #16230, #14852, #29047, #72155, #72604, #73067, #52204, #59803, #65986, #81086, #45081, #9098, #36607, #65526, #58407, #39367, #54526, #18545, #89560, #68283, #53124, #61652, #3887, #67819, #25643 ),
 ( #45539, #75842, #83395, #31372, #24730, #3405, #47413, #76322, #53612, #32297, #82004, #90485, #32764, #2944, #11448, #61202, #74440, #52656, #90038, #82483, #40300, #10498, #46940, #16684, #25190, #69215, #81536, #31830, #4344, #9572, #89098, #88644, #33221, #54063, #10965, #18086, #17161, #23792, #24250, #17630, #38459, #60261, #38910, #82934, #67365, #46026, #2495, #39833, #74929, #10040, #60721, #46482, #75385, #68756, #33691, #85749, #20896, #5762, #41230, #70634, #83878, #26112, #19029, #6709, #47883, #55006, #62117, #49307, #77730, #91906, #78201, #71094, #76787, #13340, #71573, #41718, #62602, #13804, #84334, #11913, #63546, #42181, #40762, #90948, #69680, #34636, #6227, #92375, #27534, #56427, #55947, #78663, #91444, #26595, #85289, #55485, #63076, #19485, #70170, #12880, #34174, #27060, #35097, #20438, #48351, #64015, #77254, #42656, #5304, #92855, #48823, #28018, #12384, #84802, #49768, #56909, #19952, #525, #30326, #36039, #50232, #93323, #64956, #36498, #44524, #44976, #7610, #72953, #51165, #29872, #16125, #1441, #36968, #64497, #43144, #57368, #8080, #23218, #73877, #14743, #72048, #44052, #7164, #73428, #65881, #52098, #8538, #65415, #15192, #87598, #28475, #29410, #80506, #58300, #87144, #59216, #50716, #990, #22294, #80052, #57, #37417, #58756, #86210, #15654, #22744, #51619, #66328, #80982, #28938, #88061, #43598, #86675, #35582, #79602, #57824, #21362, #79135, #14284, #21840, #72494, #3782, #9459, #8995, #9936, #61552, #54422, #38345, #83293, #3298, #10862, #88994, #1909, #24141, #60617, #67258, #82377, #39724, #68648, #82830, #2390, #53963, #17983, #90386, #31726, #38810, #47297, #89455, #24615, #37873, #31268, #10396, #17049, #32188, #61094, #52554, #66779, #89933, #60155, #81897, #74336, #32665, #53019, #75277, #46377, #25089, #45915, #74821, #25541, #30799, #67714, #59698, #46835, #68176, #88541, #53501, #75737, #2844, #23690, #81430, #17527, #39261, #18440, #16579, #45435, #40197, #48248, #48722, #33582, #12280, #85184, #26959, #19850, #33119, #63442, #13240, #18924, #41125, #40656, #27429, #63912, #5198, #70056, #20794, #34071, #91807, #76214, #69575, #77624, #84234, #5659, #34534, #26005, #11343, #92273, #76680, #55382, #47778, #42076, #11805, #12773, #41615, #70536, #26492, #4704, #6124, #69114, #91330, #62008, #56320, #20333, #4239, #55850, #49203, #62973, #90843, #54889, #77150, #62490, #78099, #70992, #83768, #19384, #84703, #34995, #92746, #27917, #56804, #85646, #87039, #6598, #36861, #80399, #86106, #14637, #14177, #886, #51057, #78560, #57263, #71467, #22189, #37314, #87951, #28835, #21255, #58195, #50125, #87489, #79945, #66222, #22639, #21735, #29300, #7968, #13698, #43495, #29769, #79501, #7508, #44416, #64850, #15083, #50611, #72391, #43039, #51511, #43943, #42550, #58647, #72840, #36393, #65777, #1336, #71941, #65306, #57719, #7062, #414, #93677, #35932, #15545, #73324, #59109, #8435, #30218, #49665, #79024, #35476, #64393, #93219, #28372, #86566, #31078, #73696, #81245, #65692, #72306, #806, #37237, #15004, #59023, #16392, #45242, #88351, #72760, #30597, #23502, #51898, #74148, #43863, #14554, #44332, #38142, #59966, #7881, #43411, #8805, #9265, #29686, #7426, #58570, #80791, #36772, #37685, #67059, #2194, #52370, #87410, #36307, #65223, #29213, #8354, #73243, #58112, #66592, #1713, #52825, #17336, #54232, #60884, #76014, #11147, #2657, #81704, #40009, #53294, #31992, #24414, #18728, #82180, #25352, #90203, #47107, #3109, #46187, #76493, #16853, #67983, #9750, #68926, #18254, #45708, #3583, #25812, #17793, #91123, #74621, #53777, #75092, #54692, #47589, #38624, #67527, #24897, #83100, #10201, #82644, #61819, #32473, #4057, #31536, #32927, #83566, #89264, #46646, #39070, #90650, #11616, #60423, #89735, #75547, #40461, #69379, #10672, #39527, #68448, #61370, #4510, #33388, #62287, #44099, #65464, #92080, #5934, #79652, #55188, #84976, #72544, #56123, #77910, #22341, #41413, #56611, #27234, #20127, #84507, #29464, #92544, #84046, #7665, #63719, #49012, #49480, #73005, #19653, #13051, #5472, #77423, #41888, #70346, #48522, #85463, #14793, #37016, #51212, #27712, #34342, #43648, #36548, #69852, #26294, #581, #26769, #63249, #91614, #87193, #55654, #20610, #58353, #80103, #70799, #12562, #15242, #19192, #34805, #76956, #8133, #65930, #48051, #12083, #40932, #4986, #33872, #62781, #1960, #59266, #2887, #60664, #22800, #58805, #66822, #67307, #52147, #30853, #9982, #45482, #38398, #51667, #81942, #31772, #37465, #59746, #88114, #45966, #2436, #29921, #8587, #80557, #31315, #82425, #39308, #73923, #66374, #9509, #1491, #38854, #60201, #17575, #67761, #88587, #74381, #53067, #87649, #23735, #74872, #52598, #81479, #89501, #16171, #89039, #16628, #24189, #23271, #24666, #17099, #15711, #53553, #46424, #75326, #10442, #1042, #81027, #44572, #9040, #45023, #73475, #37918, #30375, #4752, #55427, #77672, #63020, #47826, #91852, #68700, #68225, #69160, #27006, #19895, #3830, #48766, #62542, #70108, #54469, #61145, #83339, #26054, #32712, #76728, #5248, #34118, #48294, #61597, #19431, #77196, #55894, #90891, #4287, #12825, #54941, #83821, #3345, #90430, #84748, #12325, #25586, #41169, #32236, #89980, #18973, #33165, #25134, #11855, #40704, #54010, #18485, #69624, #76265, #91384, #26540, #18031, #82877, #84280, #47348, #11392, #39775, #46885, #40244, #33632, #75787, #10907, #62056, #35044, #65359, #5706, #56855, #92322, #64902, #7111, #34582, #86156, #14689, #6650, #79996, #41664, #42601, #6175, #43544, #7559, #63491, #27477, #13753, #14228, #92798, #71516, #50663, #21307, #79076, #56369, #28883, #72441, #78149, #35530, #63958, #86617, #43089, #70581, #49254, #85233, #71993, #29355, #20384, #20842, #13287, #50180, #42124, #79549, #35982, #58247, #36444, #64443, #3, #57771, #71041, #93269, #21787, #28423, #57314, #466, #85696, #87090, #22239, #51110, #27966, #49713, #78608, #43996, #88937, #52498, #44922, #38285, #60559, #73371, #73824, #88002, #66269, #8937, #30266, #8483, #45375, #2334, #24551, #9879, #88486, #38755, #15593, #15133, #16068, #67659, #89397, #44466, #53435, #9401, #16989, #1384, #8017, #59158, #66722, #37362, #23633, #45854, #23155, #2785, #72893, #52039, #65829, #67198, #74278, #36911, #59639, #81839, #37815, #936, #29815, #1850, #80925, #74760, #31666, #58696, #87540, #30737, #81375, #16524, #31213, #24086, #60098, #52962, #22687, #51560, #80448, #25035, #47241, #46777, #33519, #83704, #17469, #89874, #10337, #54826, #69987, #26895, #61498, #53906, #90785, #82774, #26430, #18866, #5127, #55323, #54363, #61948, #40599, #46319, #76153, #62425, #18384, #40140, #77084, #3723, #47723, #83237, #11286, #75678, #84173, #76623, #75223, #91266, #25945, #69056, #11746, #34004, #10803, #4185, #90330, #39665, #33059, #32609, #68587, #69513, #4644, #91744, #12215, #19321, #41061, #17926, #82319, #48183, #62908, #39204, #25484, #68116, #3242, #32132, #61028, #48656, #42011, #13633, #85113, #35406, #86497, #21660, #35866, #49139, #6994, #64783, #43426, #78495, #85582, #344, #42484, #71397, #55783, #20263, #57196, #63845, #78953, #14103, #5598, #84636, #42967, #56253, #34930, #27364, #50536, #78036, #28306, #93152 ),
 ( #13176, #79434, #14570, #86037, #92677, #64326, #77557, #19785, #12706, #41546, #70470, #34472, #63378, #71872, #6530, #20729, #93608, #28766, #92208, #57649, #65238, #21186, #70927, #7442, #6058, #27847, #50057, #72321, #56736, #49599, #36324, #1727, #16406, #30614, #8819, #88365, #23034, #45728, #29701, #58584, #37699, #15018, #30152, #29231, #8369, #44808, #1270, #59035, #9278, #66605, #87423, #59516, #65708, #74638, #37250, #52384, #15952, #2210, #15476, #72774, #81720, #23515, #58126, #87882, #23969, #22571, #43877, #86971, #51445, #51913, #38161, #38640, #80804, #81261, #73709, #45258, #9765, #88821, #74162, #67076, #52843, #16869, #31094, #59982, #80333, #67543, #22125, #66154, #50993, #79878, #7899, #36788, #820, #44347, #73257, #18268, #54707, #24430, #76035, #33403, #60443, #10686, #62302, #82197, #3127, #2672, #46202, #31551, #83584, #32007, #75564, #67999, #91142, #60905, #68941, #40025, #90667, #46660, #89753, #26309, #89279, #17807, #53312, #25827, #61834, #17351, #47122, #69394, #61385, #40945, #75107, #3601, #24913, #4527, #55204, #10217, #39085, #68466, #4072, #53790, #32488, #11631, #11164, #32942, #82658, #18747, #84059, #39544, #90218, #25367, #47605, #76508, #54247, #83117, #40477, #19207, #48066, #76970, #12099, #77437, #78382, #12581, #13987, #42371, #86389, #42848, #41901, #49493, #28199, #5004, #34819, #21077, #5947, #27728, #64674, #84989, #6410, #70815, #63732, #34358, #71764, #71283, #33887, #49948, #13523, #92557, #93042, #21540, #63263, #56625, #49027, #27250, #85475, #20144, #92094, #35285, #57087, #79328, #93501, #64213, #28656, #70360, #69866, #20622, #57544, #50423, #5485, #14465, #85927, #6887, #56136, #62795, #77923, #78841, #13065, #35761, #91630, #26783, #55670, #84521, #19668, #48536, #41428, #66053, #73140, #81613, #1166, #58930, #43322, #7791, #44703, #51339, #66503, #1622, #30505, #59400, #36676, #45154, #72671, #44231, #65134, #14915, #87319, #8715, #7334, #43770, #9172, #88254, #30989, #65598, #711, #22467, #59876, #30049, #29596, #66959, #2098, #80692, #80233, #51800, #235, #36214, #29115, #72218, #58011, #86867, #22021, #23412, #87780, #8266, #52278, #81157, #50891, #16301, #52730, #22930, #79772, #88716, #58475, #15369, #73604, #74053, #37146, #15846, #37592, #38050, #23864, #18163, #90113, #75919, #10578, #33296, #17237, #46099, #25265, #2567, #17705, #16762, #89634, #32378, #82557, #46558, #90559, #54142, #75004, #83011, #53201, #62194, #24804, #39914, #3485, #83472, #3018, #60335, #69289, #47016, #45616, #75457, #11525, #10116, #31446, #74517, #38982, #39441, #25717, #26193, #68357, #11044, #61279, #68835, #91024, #76403, #3963, #32837, #40372, #4418, #61727, #54601, #67895, #18628, #47494, #53690, #55087, #9652, #67440, #38537, #89172, #24324, #82079, #31904, #60796, #11989, #63624, #20969, #47960, #91985, #49836, #69757, #84412, #83956, #78733, #49386, #64569, #13876, #20029, #34710, #42729, #71644, #84878, #92449, #48426, #56980, #92933, #63154, #6777, #27612, #40838, #76864, #56509, #77808, #35654, #5838, #42260, #4888, #85368, #93394, #33772, #27138, #28546, #62685, #19560, #19105, #91518, #78278, #71174, #13416, #77331, #85818, #12464, #48906, #26674, #55564, #34248, #6303, #41311, #70248, #5383, #35171, #56023, #12958, #41796, #70707, #20518, #64093, #28094, #81044, #16187, #1057, #36566, #65946, #79210, #21431, #14353, #1977, #43213, #50305, #57437, #44588, #73021, #87208, #73492, #66390, #72114, #8603, #66842, #37032, #123, #9055, #79668, #7230, #58821, #37480, #36105, #86278, #65023, #29936, #1506, #87666, #22816, #51685, #51230, #73940, #57891, #86747, #80574, #29006, #58367, #21909, #65481, #8149, #29481, #22356, #30392, #15727, #50783, #59284, #14809, #37933, #598, #88130, #44118, #23288, #43664, #72559, #45038, #52161, #7681, #80118, #15257, #31331, #45497, #88603, #60218, #31787, #41077, #41564, #2904, #69528, #46441, #26446, #30868, #19336, #89057, #9999, #2455, #91759, #24206, #4660, #33533, #55337, #74888, #53083, #55799, #23751, #45983, #81496, #84188, #91281, #52614, #75343, #5143, #89521, #70486, #59762, #60681, #81961, #34021, #26911, #16643, #74399, #24685, #62439, #17118, #53568, #70002, #11760, #48198, #9529, #77100, #62924, #67323, #82443, #38871, #12231, #84651, #38414, #67777, #17591, #19803, #48671, #40612, #77572, #12722, #14121, #13193, #43443, #71891, #22141, #72339, #71414, #78970, #57668, #34489, #64346, #50553, #35424, #57213, #360, #20745, #35884, #6546, #93172, #63861, #7458, #7012, #63395, #79450, #42985, #28324, #28783, #51009, #92694, #86054, #78511, #56756, #21203, #49616, #27864, #64801, #86514, #15034, #29247, #93625, #58142, #6074, #5614, #50075, #86988, #79896, #34948, #43894, #21677, #36340, #85598, #92225, #13649, #14586, #42501, #65255, #27381, #56270, #85130, #20282, #49157, #78052, #42028, #70943, #8839, #17371, #30635, #88384, #72791, #37266, #74181, #80821, #2230, #31113, #22588, #37717, #23989, #66623, #59534, #67562, #87901, #9299, #73727, #44824, #66172, #74659, #45278, #7915, #52862, #16426, #1747, #60000, #24452, #1288, #23534, #51931, #30170, #52403, #23053, #59053, #38181, #88839, #82217, #2691, #81280, #31572, #73274, #36805, #67096, #60462, #53331, #8387, #65726, #81740, #9783, #15970, #837, #16890, #45747, #38658, #89297, #29719, #58601, #87442, #51463, #80352, #15493, #44364, #18286, #25385, #48084, #47142, #76052, #46223, #46681, #61853, #61404, #54725, #83601, #60925, #75127, #47623, #75584, #90236, #17829, #62322, #10704, #90684, #32960, #18765, #32507, #39562, #26327, #39105, #3620, #32028, #76526, #11649, #68017, #68958, #4545, #11182, #10237, #3146, #40042, #54265, #19226, #89772, #68484, #82679, #4089, #40496, #83135, #25844, #84076, #69414, #33420, #91162, #55222, #24934, #53811, #2067, #1593, #82051, #38507, #66026, #44675, #58903, #9620, #24776, #75431, #16273, #73577, #45583, #8686, #74975, #67411, #53659, #10087, #9142, #16730, #89146, #1138, #2540, #30958, #82528, #37565, #66476, #74488, #22901, #38019, #37117, #45124, #52701, #66929, #59846, #17208, #31419, #30475, #60308, #59371, #17676, #74025, #24295, #23835, #38955, #23379, #80662, #89606, #53171, #30020, #88687, #31876, #88223, #51772, #87749, #52248, #81582, #46069, #46529, #67867, #2990, #60765, #15818, #81129, #70216, #40343, #55054, #5350, #34216, #11494, #83923, #68803, #77298, #19529, #83440, #41279, #19075, #61248, #68330, #47929, #4389, #63122, #26162, #62652, #32349, #76832, #91951, #3454, #18595, #27106, #90083, #11012, #10549, #55990, #69724, #91487, #33739, #3932, #12428, #39882, #69260, #25235, #75886, #54570, #4855, #54109, #32806, #84845, #26641, #19993, #61696, #90528, #47461, #48872, #62163, #25688, #39414, #82982, #11959, #76368, #40807, #18132, #46986, #33266, #90992, #55531, #84380, #48395, #64994, #93362, #13845, #97, #86717, #70675, #28976, #87181, #57407, #20484, #29451, #6268, #92416, #79178, #57861, #41764, #12923, #27576, #50269, #21882, #14323, #86247, #49807, #21398, #36076, #5804, #42696, #50754, #71615, #35622, #72531, #92901, #43183, #78703, #6749, #42225, #79638, #72085, #34678, #14780, #7201, #64537, #43633, #58339, #71139, #28513 ),
 ( #7650, #36535, #64059, #56474, #65450, #566, #63592, #22330, #77776, #78245, #85333, #49350, #13382, #35136, #28060, #56950, #85787, #20938, #66813, #45472, #31762, #17085, #81016, #1943, #45954, #74860, #52136, #30841, #15698, #24178, #60191, #30363, #81932, #59735, #8120, #15231, #88577, #45012, #9972, #23725, #9496, #72990, #52588, #38844, #44087, #59252, #67751, #37006, #51655, #51201, #2877, #16618, #38384, #74372, #44560, #53057, #80541, #16160, #65919, #22786, #1478, #67297, #1031, #73463, #60654, #2425, #89491, #8575, #37453, #88098, #80089, #9030, #66362, #29909, #58793, #81469, #23258, #31305, #87637, #73913, #37908, #89029, #18475, #39762, #82868, #54926, #11841, #34107, #19420, #4276, #48282, #25125, #24652, #25576, #77185, #70093, #53999, #5235, #18961, #26528, #10897, #17562, #68688, #76253, #18021, #33154, #55417, #84269, #4740, #46874, #69611, #33620, #12314, #47335, #54458, #63009, #11382, #40233, #53541, #75777, #26042, #32701, #47814, #76715, #68216, #82415, #40692, #3820, #61587, #89971, #41158, #90419, #90879, #62045, #62527, #83329, #69148, #46414, #75315, #83808, #10433, #91369, #39298, #3336, #32225, #61134, #56841, #36428, #91840, #92782, #56355, #93712, #57755, #19884, #55883, #63944, #64428, #49241, #27951, #7096, #42586, #35513, #48755, #79061, #28867, #34569, #85682, #85217, #43073, #93254, #26995, #5694, #77660, #28408, #79535, #84736, #71027, #63478, #6633, #92307, #35967, #57299, #14674, #64887, #20829, #71501, #50164, #12812, #49698, #71977, #78594, #13736, #86601, #13274, #86141, #21291, #14212, #20370, #21770, #50646, #41652, #43530, #72427, #7544, #70569, #27463, #78136, #42111, #6160, #35030, #59622, #22673, #38270, #16509, #16974, #88921, #23140, #44906, #45839, #29337, #52022, #58231, #80908, #87075, #22224, #51093, #43980, #39648, #10787, #3226, #40583, #11271, #67644, #18850, #76137, #68571, #61933, #84158, #32117, #3708, #17910, #89859, #32593, #53891, #61013, #69041, #25928, #48167, #33502, #18367, #62409, #39189, #38739, #61483, #91251, #19306, #68101, #77069, #33043, #69498, #25019, #31652, #82758, #90315, #46762, #47227, #4629, #26415, #47708, #75663, #83689, #76607, #55305, #25468, #54348, #2769, #83222, #40124, #60542, #4170, #90769, #54811, #11731, #89380, #82302, #24535, #53419, #17453, #46303, #10321, #75207, #41530, #78479, #49584, #6513, #56235, #5583, #35851, #69971, #27349, #62892, #35391, #71379, #5111, #56721, #78935, #70909, #50521, #12200, #13160, #70456, #14086, #71857, #33989, #91728, #78020, #13616, #63362, #41996, #21171, #85567, #42469, #26881, #93136, #42951, #48638, #6043, #34454, #57181, #64311, #41043, #19769, #55767, #28291, #93592, #21643, #20714, #77540, #57634, #92193, #84621, #86021, #50040, #12690, #85098, #20248, #6978, #64768, #28751, #86477, #49124, #34915, #63827, #92660, #27832, #76135, #53417, #3706, #67642, #75661, #83220, #39646, #90313, #47706, #11269, #68099, #40122, #10319, #84156, #10785, #25926, #54346, #40581, #53889, #17451, #26413, #69039, #31650, #25466, #62407, #3224, #82300, #60540, #32115, #18365, #76605, #77067, #47225, #4168, #33041, #61931, #48165, #33500, #54809, #83687, #91249, #55303, #18848, #11729, #61011, #69496, #4627, #19304, #12198, #89378, #46301, #75205, #39187, #89857, #25017, #82756, #17908, #62890, #20712, #71855, #5109, #49122, #6976, #26878, #41528, #41041, #35849, #6511, #28289, #64309, #34452, #42949, #70454, #41994, #91726, #12688, #85096, #35389, #33987, #5581, #64766, #57179, #28749, #63360, #92191, #20245, #57632, #92658, #27347, #93590, #86475, #78477, #78018, #49582, #55765, #84619, #19767, #79418, #48636, #77538, #69969, #86019, #56719, #70907, #21169, #50038, #56233, #78933, #13158, #21641, #6041, #13614, #42467, #93134, #34913, #63825, #50519, #27830, #85565, #71377, #14084, #73693, #72304, #59021, #81243, #73241, #52822, #14552, #15458, #72758, #16390, #74146, #36305, #7424, #80319, #80789, #65690, #44330, #23500, #87869, #51896, #65221, #1711, #45240, #50978, #8352, #7879, #59498, #15938, #43409, #22109, #326, #44792, #2192, #29211, #87408, #79863, #23018, #15002, #52368, #8803, #31076, #9263, #37235, #37683, #66590, #58110, #66140, #88349, #1256, #30137, #38140, #29684, #30595, #67057, #59964, #36770, #88803, #23950, #86956, #43861, #804, #58568, #22555, #51430, #46185, #17791, #60882, #39068, #75545, #3107, #75090, #18252, #68924, #91121, #76491, #61368, #11614, #82178, #81702, #82642, #40459, #33386, #17334, #62285, #76012, #83564, #67981, #74619, #31990, #39525, #10199, #90201, #18726, #47587, #61816, #89733, #32925, #90648, #69377, #10670, #46644, #26292, #68446, #3581, #16851, #24895, #83098, #53775, #11145, #40007, #31534, #45706, #4055, #32470, #25350, #4508, #9748, #25810, #54230, #54690, #38622, #67525, #47105, #2655, #60421, #89261, #24412, #53292, #19651, #56609, #63247, #78369, #13508, #4984, #55186, #42356, #55652, #34340, #26767, #21064, #84505, #27710, #92542, #49478, #5470, #48520, #78828, #19190, #70344, #12081, #71270, #20608, #48049, #5932, #28185, #20125, #93489, #84044, #56121, #77421, #57074, #49931, #76954, #40930, #27232, #85461, #12560, #84974, #64198, #34803, #6397, #69850, #35269, #85912, #91612, #49010, #41411, #93029, #13974, #33870, #62779, #92078, #42832, #71749, #77908, #13049, #41886, #63717, #70797, #6875, #35748, #64661, #66491, #699, #8252, #80677, #57531, #87306, #73591, #58462, #80218, #23398, #43757, #58917, #29583, #22453, #86852, #30493, #1153, #86376, #8702, #66041, #51326, #51787, #74040, #22008, #15357, #7778, #79760, #44217, #72656, #50878, #87764, #15833, #38037, #52264, #37133, #81144, #29102, #28642, #73125, #16288, #9157, #57996, #66945, #22917, #59387, #14902, #21527, #36664, #30036, #65584, #44690, #37580, #1607, #50407, #88239, #45141, #79313, #14452, #43309, #72205, #7322, #36200, #65119, #222, #27005, #55893, #40703, #76264, #11854, #23851, #59862, #52717, #41663, #81599, #88703, #2084, #84279, #18972, #33164, #19430, #12324, #18030, #48293, #12824, #76727, #39774, #48765, #25585, #46884, #4751, #77195, #75786, #30974, #10906, #69623, #41168, #33631, #62541, #91383, #90890, #19894, #3829, #32711, #26539, #68699, #4286, #61596, #11391, #47825, #69159, #62055, #70107, #55426, #90429, #5247, #54468, #77671, #40243, #34117, #83820, #63019, #83338, #18484, #84747, #91851, #47347, #26053, #54940, #71040, #85232, #34581, #6174, #71515, #79548, #79995, #42600, #14227, #86155, #64901, #51109, #36443, #6649, #21306, #65358, #465, #35529, #50179, #35043, #43543, #14688, #49712, #7558, #79075, #27476, #63490, #43088, #64442, #29354, #71992, #28882, #92321, #7110, #58246, #56368, #78607, #87089, #20383, #63957, #70580, #22238, #35981, #57770, #2, #92797, #72440, #27965, #93268, #49253, #42123, #78148, #86616, #15132, #13286, #13752, #5705, #56854, #85695, #20841, #28422, #21786, #50662, #57313, #37361, #45853, #73370, #44921, #65828, #15592, #88001, #9400, #8016, #44465, #9878, #31212, #31665, #8482, #66268, #23154, #60557, #1849, #1383, #67658, #2784, #81374, #52038, #52497, #935, #36910, #29814, #82317, #58695, #87539, #43995, #60097, #59638, #73823, #88936, #52961, #22686, #24085 ),
 ( #8936, #89395, #24549, #30265, #53433, #38284, #74759, #59157, #51559, #80924, #30736, #16067, #23632, #38754, #72892, #81838, #37814, #16988, #80447, #66721, #88485, #16523, #45374, #74277, #67197, #2333, #75676, #18864, #25482, #40597, #69511, #61026, #17467, #4642, #17924, #90328, #82772, #77082, #46775, #83702, #54824, #11744, #61496, #10801, #41059, #75221, #32607, #68114, #33517, #76621, #10335, #61946, #84171, #54361, #62423, #4183, #19319, #3721, #89872, #69985, #47721, #46317, #76151, #12213, #39663, #32130, #39202, #68585, #18382, #26428, #26893, #83235, #91264, #33057, #55321, #91742, #5125, #47239, #90783, #34002, #62906, #11284, #25943, #40138, #48181, #55781, #69054, #3240, #25033, #53904, #48654, #35404, #78493, #21658, #6528, #42965, #12704, #64324, #50534, #77555, #92675, #79432, #70468, #85111, #84634, #14568, #50055, #71870, #14101, #78034, #86495, #20261, #85580, #41544, #56251, #34928, #78951, #5596, #49137, #43424, #6992, #72319, #13174, #42009, #63843, #7440, #42482, #70925, #36322, #65236, #28304, #27845, #93150, #34470, #63376, #92206, #29229, #27362, #6056, #19783, #35864, #57194, #20727, #64781, #93606, #56734, #28764, #342, #86035, #49597, #13631, #71395, #21184, #57647, #45255, #22123, #86969, #72772, #30611, #74159, #59513, #37696, #23512, #51911, #74635, #58582, #87421, #66602, #43875, #59033, #58124, #37248, #73706, #30150, #87880, #38158, #1724, #22569, #88362, #818, #9762, #52381, #66152, #81258, #79876, #50991, #15016, #2669, #7897, #36786, #65706, #9275, #8816, #23032, #67073, #2207, #29699, #31091, #67540, #16403, #51443, #38637, #80331, #15474, #59979, #88818, #44345, #73255, #8367, #23966, #52840, #81717, #16866, #45725, #80802, #1268, #15950, #44805, #54244, #82194, #10683, #31548, #46657, #90215, #39541, #68463, #90664, #83114, #3124, #47119, #39082, #69391, #75561, #68938, #25364, #83581, #53787, #75104, #40474, #76032, #89276, #3598, #76505, #67996, #17348, #24427, #32004, #32485, #25824, #62299, #61382, #18265, #11161, #40022, #60440, #4524, #4069, #32939, #33400, #53309, #61831, #54704, #17804, #46199, #10214, #18744, #60902, #47602, #11628, #24910, #89750, #82655, #53150, #38000, #74468, #44187, #2048, #82031, #80187, #30457, #17189, #8222, #22885, #22423, #46051, #81561, #9599, #45564, #15799, #24275, #51754, #23361, #73092, #87733, #66457, #16709, #15326, #80644, #74956, #38486, #10067, #44658, #73559, #1575, #38936, #74006, #8668, #67845, #2971, #30002, #60287, #88668, #31856, #89124, #88203, #30938, #67391, #51295, #81111, #2520, #52228, #9123, #60745, #37546, #52680, #16254, #45104, #59352, #37100, #23817, #66009, #31397, #59827, #66910, #1121, #58887, #54089, #25671, #68783, #46966, #83419, #10992, #82960, #26139, #76813, #5330, #84359, #69240, #19509, #90064, #89586, #90509, #48377, #41258, #25216, #70197, #83903, #91469, #75868, #82509, #39861, #47439, #18114, #4369, #26620, #55511, #69705, #3912, #40787, #4835, #77279, #18574, #54551, #34198, #76348, #11474, #24757, #32789, #90973, #61677, #19054, #47910, #39394, #53639, #11938, #40325, #33247, #61229, #12408, #62143, #55034, #33719, #62630, #17657, #46509, #75411, #10527, #68309, #3432, #32327, #28495, #27085, #13825, #36058, #28042, #7632, #63102, #64038, #27558, #64976, #28957, #84825, #55972, #35118, #35603, #20464, #92880, #72066, #42677, #6730, #19974, #50251, #79, #5784, #56932, #56453, #14305, #64518, #91930, #70656, #48850, #93344, #50736, #77755, #42205, #34658, #71594, #12904, #85769, #41743, #71119, #78685, #20919, #49788, #43165, #57388, #63572, #86230, #92398, #79620, #6249, #21381, #79157, #57843, #49331, #85315, #21862, #7183, #78225, #86697, #14762, #13364, #43616, #72512, #36987, #37436, #45455, #45934, #8556, #73895, #52117, #30820, #17067, #2408, #66345, #80999, #31288, #60174, #1459, #16142, #1011, #9478, #74355, #15677, #67278, #44994, #87163, #546, #9012, #30345, #89012, #37891, #88560, #58319, #66796, #24159, #29429, #44543, #53039, #22312, #65899, #36517, #81915, #1926, #23708, #59717, #29891, #38364, #58775, #59235, #51183, #8100, #80524, #52571, #80070, #87617, #74842, #81451, #65432, #22768, #51638, #73446, #15213, #88081, #23237, #44069, #72971, #16599, #82851, #18458, #31743, #67734, #60636, #48266, #89473, #2860, #9955, #90862, #25560, #39743, #26026, #18943, #24634, #54909, #19403, #83313, #46397, #55400, #32207, #53521, #11364, #83788, #82397, #38827, #17545, #76233, #47797, #40216, #47317, #69132, #3803, #26511, #10416, #39280, #4260, #75297, #33138, #76699, #68198, #3318, #61114, #62028, #11825, #40676, #69594, #4724, #32684, #84252, #89953, #25108, #33602, #53982, #10880, #18003, #46856, #54440, #75759, #68667, #62510, #91350, #61570, #90403, #19868, #93696, #85200, #6615, #63927, #50145, #63459, #26976, #35951, #49682, #12298, #42094, #71960, #77642, #91823, #41142, #12793, #78119, #86124, #86583, #49222, #20812, #92765, #71483, #57738, #43056, #13257, #27932, #7078, #64870, #71009, #56823, #41634, #79043, #21273, #56338, #14195, #85664, #34090, #70075, #78577, #6140, #28852, #13715, #35495, #5217, #42567, #21753, #62992, #20350, #77168, #55867, #70553, #84719, #48738, #64410, #93237, #28390, #5676, #34551, #92289, #35012, #27446, #57282, #904, #16037, #14658, #51076, #16491, #37784, #38253, #15101, #79964, #29786, #67166, #8451, #22206, #74247, #9369, #87970, #58665, #59126, #72411, #43513, #7527, #88905, #36412, #65328, #50629, #66691, #66238, #80418, #1819, #59604, #432, #30705, #60068, #30236, #87057, #2299, #72860, #44890, #87509, #43961, #31182, #29320, #65794, #58212, #73791, #8907, #7985, #1353, #23601, #15563, #79519, #36879, #51529, #22656, #52469, #45345, #44434, #73340, #37330, #23121, #52004, #80890, #88454, #81343, #61472, #74728, #11255, #54795, #60527, #82743, #82287, #69025, #25454, #52929, #31637, #45822, #90302, #11715, #62393, #3211, #89363, #32579, #24521, #61918, #54333, #40568, #90754, #89844, #3694, #76123, #81808, #17896, #4157, #53877, #75650, #18836, #39175, #83207, #25006, #46749, #17438, #25912, #18354, #16957, #33027, #47212, #10773, #40110, #69483, #46288, #39633, #32097, #75192, #68557, #68086, #10305, #83674, #47691, #33487, #76593, #4613, #24055, #53402, #9849, #38722, #67628, #2756, #60999, #44203, #86833, #682, #78814, #84143, #13960, #50391, #26864, #72190, #29567, #58447, #72642, #85899, #43742, #7763, #80203, #21513, #28628, #37116, #79295, #14436, #91236, #55752, #207, #6858, #21991, #50864, #41027, #26401, #79746, #91712, #71731, #62878, #87292, #21051, #65105, #36186, #33974, #73110, #49918, #12184, #29088, #14888, #55289, #19292, #69953, #57981, #36648, #65569, #7307, #22438, #86361, #15342, #42817, #35733, #51311, #77055, #93475, #48151, #64646, #43293, #57517, #8237, #5095, #74486, #66474, #38505, #8685, #82526, #74023, #89144, #52699, #38953, #52246, #15817, #24774, #67409, #1137, #30956, #60763, #1591, #80661, #30019, #30473, #66927, #74973, #75429, #38017, #9618, #81580, #60306, #46527, #31874, #2065, #16728, #89604, #53657, #59844, #45581, #59369, #67865, #10085, #45122, #2988, #2538, #22900, #58902, #31417, #88685, #17674, #24293, #53169, #87748, #82049 ),
 ( #51771, #17206, #10547, #66025, #9140, #73576, #46067, #37564, #44674, #88221, #23377, #81127, #23833, #16271, #26639, #68328, #4387, #84378, #69258, #90990, #34214, #54568, #69722, #40341, #11492, #3930, #33264, #62650, #84843, #32804, #62161, #18593, #90526, #26160, #83438, #61694, #4853, #55529, #48870, #63120, #19073, #91949, #39880, #39412, #55052, #27104, #19991, #68801, #77774, #33737, #41277, #47459, #32347, #76366, #83921, #47927, #76830, #70214, #5348, #19527, #11957, #48393, #77296, #55988, #40805, #12426, #3452, #61246, #90081, #25233, #54107, #82980, #18130, #46984, #75884, #11010, #12921, #95, #13380, #85785, #78243, #72529, #42223, #79176, #50267, #7199, #56948, #6266, #36533, #70673, #28058, #63590, #36074, #72083, #5802, #57405, #79636, #71613, #51199, #41762, #13843, #71137, #14778, #7648, #34676, #92414, #78701, #14321, #64057, #42694, #21880, #86245, #43181, #27574, #28974, #43631, #49348, #6747, #35134, #57859, #64992, #56472, #20482, #85331, #86715, #564, #92899, #20936, #49805, #21396, #35620, #50752, #65448, #29449, #58337, #64535, #87179, #22328, #93360, #28511, #31304, #16159, #37907, #74859, #1477, #16617, #81015, #52135, #44559, #81931, #52587, #15229, #60190, #23724, #1942, #80087, #73462, #81468, #88097, #9495, #38383, #29907, #44085, #67296, #80540, #59251, #51654, #45953, #15697, #45471, #74371, #2424, #30362, #8574, #9971, #72988, #23257, #37004, #89028, #24177, #8118, #30840, #53056, #45011, #24651, #65917, #73912, #37452, #17084, #38843, #1029, #58791, #9029, #67750, #66361, #66812, #2876, #59734, #31761, #87636, #60653, #89490, #22785, #88576, #18020, #4739, #54925, #82414, #61133, #75314, #26041, #41157, #91839, #32700, #89970, #62044, #25124, #91368, #83806, #70092, #26527, #25575, #33153, #11840, #17561, #18474, #33619, #83328, #11381, #48281, #68687, #18960, #54457, #47334, #46873, #55416, #47813, #46413, #62526, #90878, #76252, #76714, #5234, #75776, #40232, #61586, #10896, #69147, #3819, #39761, #40691, #69610, #63008, #77184, #84268, #12313, #53998, #53540, #4275, #34106, #10432, #82867, #39297, #19418, #68215, #90418, #3335, #32224, #78593, #56354, #6632, #57754, #86600, #7095, #20369, #71976, #35966, #14673, #49697, #56840, #65344, #13735, #21290, #71026, #49240, #50645, #84735, #42110, #77659, #50163, #86140, #19883, #71500, #93711, #85681, #26994, #55882, #27950, #85216, #28866, #21769, #48754, #12811, #92781, #93253, #78135, #20828, #64886, #35512, #64427, #41651, #14211, #79534, #63477, #42585, #13273, #43529, #28407, #70568, #34568, #5693, #57298, #72426, #92306, #6159, #27462, #79060, #35029, #7543, #43072, #36427, #63943, #66253, #73807, #52483, #29335, #59142, #45359, #30251, #52020, #88919, #15579, #30721, #1369, #87986, #58681, #2315, #66705, #58230, #74262, #37799, #23138, #23616, #45837, #87526, #80906, #73355, #51545, #16052, #44449, #22672, #59620, #81357, #9863, #24069, #8921, #52945, #921, #451, #44904, #81822, #74742, #29800, #38737, #88469, #31197, #80434, #87074, #8467, #1834, #37347, #16507, #60082, #16972, #9385, #38268, #67181, #22223, #51092, #79981, #15118, #43979, #72878, #8002, #36894, #65810, #93346, #6251, #21383, #79159, #5786, #91932, #43167, #49333, #71121, #63574, #57845, #78227, #64520, #35605, #84827, #13827, #86699, #13366, #12906, #19976, #42207, #92882, #7185, #7634, #64040, #28497, #71596, #72068, #72514, #50738, #36060, #28959, #79622, #14764, #48852, #77758, #34660, #38366, #74357, #44545, #2410, #16144, #22314, #29431, #44996, #59237, #31290, #81001, #23710, #87165, #73897, #60176, #58321, #73448, #89014, #51185, #65901, #65434, #24161, #30822, #52573, #88562, #58777, #67280, #1013, #66347, #80072, #36989, #15679, #59719, #15215, #29893, #53041, #81453, #81917, #87619, #22770, #8558, #17069, #23239, #51640, #45936, #74844, #9014, #37437, #37893, #44071, #72973, #8102, #9957, #80526, #1461, #548, #16601, #66798, #30347, #45457, #9480, #88083, #52119, #1928, #18460, #75299, #84254, #61116, #53523, #40218, #26028, #2862, #67736, #82399, #11366, #54911, #69134, #47319, #4262, #32686, #55402, #39282, #68200, #76235, #24636, #39745, #38829, #18005, #54442, #10882, #68669, #18945, #33140, #3320, #62030, #10418, #19405, #46858, #90864, #25562, #11827, #25110, #17547, #91352, #83790, #32209, #3805, #60638, #89955, #82853, #47799, #31745, #53984, #4726, #76701, #26513, #75761, #61572, #90405, #48268, #83315, #40678, #62512, #77170, #69596, #33604, #89475, #46399, #70077, #34092, #50631, #62994, #5219, #12300, #93239, #27934, #42096, #28392, #21275, #91825, #57284, #21755, #85666, #48740, #57740, #34553, #26978, #13717, #86126, #55869, #41144, #84721, #78579, #50147, #42569, #20814, #71485, #6142, #28854, #12795, #41636, #49684, #19870, #13259, #77644, #85202, #56825, #78121, #71011, #79045, #6617, #70555, #35497, #5678, #86585, #20352, #64412, #92767, #14197, #92291, #63461, #64872, #43058, #27448, #35014, #7080, #56340, #49224, #63929, #71962, #35953, #93698, #88907, #51531, #23123, #1355, #73793, #60070, #45347, #15565, #30238, #74249, #9371, #80420, #59128, #43963, #52471, #88456, #58667, #16493, #87972, #36414, #43515, #52006, #73342, #38255, #80892, #37786, #7529, #16039, #67168, #72413, #87511, #2301, #65330, #79966, #79521, #31184, #44892, #66693, #8909, #72862, #81345, #1821, #29788, #7987, #24057, #434, #906, #29322, #30707, #59606, #58214, #23603, #14660, #44436, #87059, #22208, #8453, #36881, #51078, #15103, #65796, #22658, #37332, #66240, #10307, #82745, #61920, #3696, #90304, #9851, #40112, #83676, #89365, #17898, #17440, #4159, #54335, #81810, #60529, #74730, #25456, #40570, #91238, #32099, #24523, #61474, #53404, #90756, #83209, #69485, #25914, #25008, #32581, #11257, #16959, #46751, #33029, #75652, #10775, #47693, #68088, #18356, #53879, #39635, #46290, #54797, #47214, #45824, #18838, #76125, #68559, #69027, #4615, #75194, #76595, #61001, #39177, #11717, #3213, #89846, #33489, #62395, #52931, #38724, #67630, #2758, #82289, #31639, #27336, #78921, #71844, #55754, #6964, #20702, #28279, #12676, #19294, #41518, #78008, #84607, #6029, #57169, #86009, #6497, #19756, #71367, #35378, #14070, #49111, #56223, #64754, #13148, #41984, #26403, #48623, #27818, #34442, #49572, #78467, #69955, #55291, #13604, #26866, #5571, #91714, #21159, #77524, #92646, #63814, #85083, #42455, #64297, #48153, #93123, #35837, #34903, #62880, #84145, #70444, #41029, #56708, #50028, #77057, #12186, #5097, #85554, #42935, #33976, #63348, #92181, #20234, #70897, #314, #29197, #8340, #79405, #790, #93579, #72746, #15447, #65678, #29672, #73680, #37221, #58094, #66128, #36293, #16378, #7867, #23005, #80308, #66579, #79850, #43396, #52355, #1243, #28738, #58553, #88336, #86944, #14541, #57621, #22096, #87397, #8791, #9251, #22544, #30125, #44316, #87856, #74133, #59483, #51418, #73228, #23488, #81231, #59009, #51883, #50966, #1699, #37670, #36756, #30582, #80776, #50507, #86464, #15926, #44780, #45228, #38129, #21625, #72291, #7412, #65210, #14989, #43848, #4047, #52812, #67516, #67042, #32917, #32458, #54220, #90192, #60412, #68916, #2646, #67970, #88792, #38613, #17323, #61358, #31065 ),
 ( #23940, #83089, #61807, #9736, #31980, #31524, #18244, #68436, #2179, #74607, #81692, #39515, #54682, #11606, #46174, #89252, #75535, #24403, #11133, #3568, #83556, #39997, #39058, #46634, #25340, #59953, #60873, #47096, #3097, #24884, #90639, #82166, #76003, #89720, #53765, #53282, #25802, #18715, #16840, #47578, #10659, #82631, #76483, #45696, #75078, #17780, #10189, #91603, #34333, #55644, #4975, #70789, #27700, #49923, #35260, #20116, #64186, #40921, #40451, #41400, #93019, #85904, #69841, #21056, #34794, #42348, #26759, #33377, #84497, #92070, #33861, #48998, #71261, #6389, #20600, #62771, #85452, #49470, #28176, #63239, #70335, #78820, #27224, #56112, #69369, #19643, #41878, #48511, #63709, #92534, #84036, #4499, #56598, #77412, #12550, #12073, #57066, #5463, #13041, #77897, #78360, #84965, #5924, #62276, #91111, #13500, #26280, #55176, #19181, #48041, #76946, #80668, #72648, #52254, #13965, #14894, #72196, #15824, #73583, #35739, #71738, #79752, #80209, #65111, #43748, #22908, #58454, #51317, #64652, #1145, #44681, #50397, #7770, #7313, #58909, #15349, #42823, #21519, #93481, #44209, #1599, #6865, #86840, #79302, #22444, #14443, #51779, #73116, #30482, #8692, #36654, #87298, #66032, #28634, #65575, #87755, #689, #29573, #37572, #29094, #8243, #37124, #30026, #36192, #66482, #59377, #57523, #88229, #23385, #86368, #43299, #214, #57987, #21999, #50870, #38513, #74981, #2546, #45591, #17683, #68337, #90535, #75895, #60772, #11019, #81588, #81135, #82057, #39889, #32813, #16736, #61703, #75437, #82989, #67417, #74031, #31425, #38961, #74494, #89612, #18139, #46993, #61254, #9626, #32355, #90090, #68810, #10093, #17214, #25695, #67873, #2996, #16279, #60314, #82534, #89152, #10555, #39420, #30964, #45130, #3460, #24301, #53178, #52707, #3939, #46075, #53665, #24783, #25242, #31882, #46535, #9148, #38026, #54116, #66935, #2073, #59852, #88693, #23841, #27586, #19536, #92907, #54577, #55538, #19082, #56483, #20492, #76375, #18603, #26648, #27114, #11966, #84387, #63600, #5358, #91959, #33747, #63130, #11501, #47468, #40350, #83448, #69267, #4396, #33273, #41772, #70223, #48402, #70682, #92424, #62170, #5812, #64067, #34224, #91001, #6275, #76839, #26170, #55998, #34686, #55061, #83930, #47936, #84853, #85341, #20003, #48881, #77784, #77305, #71146, #40814, #69731, #12932, #4864, #12437, #62659, #91493, #49358, #41288, #78252, #13390, #42233, #35144, #1835, #64543, #45838, #37348, #52484, #16053, #2317, #14329, #71622, #81823, #30722, #56956, #87987, #24070, #28519, #42704, #85793, #57414, #30252, #38269, #38738, #1370, #66706, #44905, #23617, #9864, #88920, #59143, #73808, #52946, #16973, #23139, #8922, #86253, #31198, #67182, #8468, #60083, #37800, #78709, #20944, #59621, #52021, #74743, #88470, #81358, #49812, #16508, #67643, #13851, #66254, #28067, #6755, #21404, #35628, #93369, #45360, #74263, #9386, #50277, #79185, #43189, #80907, #73356, #68100, #46761, #61932, #60541, #3225, #62408, #83688, #84157, #61012, #32116, #75662, #19305, #54347, #89858, #26414, #55304, #40123, #90768, #10786, #25018, #48166, #89379, #17909, #53418, #25927, #54810, #24534, #47226, #69497, #61482, #41042, #2768, #3707, #53890, #4628, #91250, #82301, #17452, #68570, #69040, #82757, #32592, #11730, #76136, #4169, #46302, #18849, #33501, #39188, #90314, #39647, #47707, #33042, #31651, #10320, #75206, #76606, #77068, #25467, #83221, #18366, #11270, #40582, #12199, #42468, #86476, #14085, #41995, #49583, #28290, #5110, #34914, #21170, #6042, #27831, #64767, #85097, #6512, #70908, #63826, #34453, #71856, #71378, #33988, #50039, #13615, #92659, #93135, #21642, #63361, #56720, #49123, #27348, #85566, #20247, #92192, #35390, #57180, #79419, #93591, #78478, #28750, #70455, #69970, #20713, #57633, #50520, #5582, #14553, #64310, #6977, #56234, #62891, #78019, #86020, #13159, #78934, #35850, #91727, #42950, #26880, #55766, #84620, #19768, #48637, #77539, #12689, #41529, #59022, #43410, #7880, #44793, #51431, #66591, #1712, #86957, #72305, #30596, #43862, #22556, #15003, #9264, #72759, #15939, #80790, #87409, #8804, #7425, #36771, #38141, #59499, #31077, #65691, #805, #80320, #59965, #1257, #29685, #67058, #2193, #73695, #15459, #51897, #65222, #36306, #327, #81703, #29212, #58111, #22110, #88350, #87870, #73242, #23501, #52369, #50979, #81244, #52824, #23019, #79864, #88804, #58569, #44331, #37684, #16391, #8353, #37236, #66141, #45241, #74147, #23951, #30138, #76013, #10671, #33387, #17335, #46186, #25351, #2656, #17792, #16852, #89734, #32472, #82643, #46645, #90649, #54231, #75091, #83099, #53293, #62286, #24896, #40008, #3582, #83565, #3108, #60422, #69378, #18253, #45707, #75546, #11615, #10200, #31535, #74620, #39069, #39526, #25811, #26293, #68447, #47106, #61369, #11146, #91122, #76492, #90202, #68925, #40460, #4509, #4056, #32926, #67982, #18727, #54691, #53776, #47588, #61818, #67526, #9749, #55187, #38623, #89263, #24413, #82179, #31991, #60883, #21065, #48050, #92079, #49932, #69851, #84506, #84045, #78829, #49479, #71271, #13509, #77422, #85913, #19652, #84975, #12082, #55653, #42357, #12561, #13975, #48521, #20126, #40931, #41412, #34341, #78370, #76955, #70345, #42833, #6398, #71750, #5471, #63248, #27233, #6876, #41887, #56122, #35749, #64662, #27711, #49011, #92543, #4985, #33871, #62780, #28643, #91613, #26768, #19191, #35270, #5933, #77909, #64199, #93030, #13050, #28186, #93490, #63718, #70798, #34804, #56610, #85462, #20609, #57075, #21528, #86377, #72206, #30037, #44691, #58918, #37134, #22918, #51327, #74041, #57997, #86853, #66042, #43310, #58463, #57532, #36665, #73126, #29584, #87307, #37581, #1154, #22009, #87765, #223, #9158, #65585, #80678, #44218, #30494, #43758, #7323, #16289, #51788, #50408, #22454, #52265, #50879, #36201, #79314, #79761, #80219, #66492, #66946, #15358, #15834, #8253, #73592, #38038, #23399, #8703, #1608, #81145, #45142, #59388, #88240, #14903, #2085, #14453, #700, #65120, #29103, #72657, #7779, #75446, #24790, #61713, #46543, #82998, #52718, #10564, #90547, #88704, #38971, #25705, #16748, #31434, #30975, #54588, #90100, #18150, #82067, #60784, #39900, #39429, #68346, #81600, #47003, #83459, #67427, #89622, #89161, #75907, #32364, #59863, #38523, #45603, #3473, #18615, #69276, #10103, #2555, #61265, #60324, #68821, #25251, #47479, #3951, #3006, #54127, #11032, #23852, #53675, #32823, #82542, #17693, #76388, #46085, #11512, #31891, #40359, #24311, #74505, #9636, #53189, #17223, #74992, #67882, #27597, #49824, #62669, #34234, #77315, #55548, #91969, #19546, #91503, #34696, #85353, #13862, #92917, #77793, #28079, #4874, #4405, #5367, #56967, #78721, #33758, #42716, #92433, #6286, #84397, #91012, #48412, #56007, #26659, #12943, #35157, #64078, #78263, #12449, #49370, #13401, #85805, #27124, #63140, #33284, #84863, #20014, #62179, #41297, #5822, #70233, #56494, #20501, #47946, #26180, #42245, #48892, #41781, #69742, #20955, #70692, #63609, #71158, #55071, #83940, #19093, #76848, #11975, #40823, #28533, #1045, #37020, #35640, #22344, #44576, #36551, #16174, #71633, #72547, #36091, #73479, #37468, #93381, #64557, #43651, #44103, #6765, #58808 ),
 ( #81030, #66377, #51215, #1494, #72101, #57425, #7669, #30378, #23275, #7218, #52149, #65934, #8591, #57880, #86266, #86735, #29468, #65012, #80106, #59269, #88117, #51670, #112, #22803, #80561, #21417, #585, #65468, #50292, #58356, #87196, #79198, #28992, #73008, #79655, #29924, #87652, #14341, #43200, #15714, #21897, #50770, #14796, #15245, #8137, #2890, #67763, #24669, #67309, #45484, #61147, #73925, #38400, #66824, #53555, #89503, #9042, #9984, #39310, #53069, #46887, #45026, #81944, #2439, #89982, #25136, #30855, #1963, #17102, #82427, #31317, #45968, #3348, #31775, #60667, #59749, #75329, #54012, #16630, #74874, #60204, #10444, #17577, #88589, #81482, #23738, #46426, #18034, #37920, #38857, #89042, #68228, #24192, #52601, #32239, #74383, #9512, #82879, #15549, #87954, #64854, #87043, #29772, #51061, #418, #66225, #23107, #45333, #30690, #44421, #59590, #36397, #35936, #36865, #88440, #81330, #65311, #16477, #30222, #37771, #22192, #28839, #79948, #87493, #29305, #73327, #66677, #1804, #16025, #58199, #80878, #44876, #23589, #58651, #65780, #74234, #22642, #51514, #93681, #15086, #37317, #43946, #59113, #51990, #79505, #57723, #73778, #72843, #7971, #7512, #52456, #889, #8438, #1339, #8893, #80402, #86570, #21739, #50615, #14642, #43499, #72395, #68543, #67152, #53865, #76111, #68074, #47680, #9354, #10292, #67616, #11244, #69014, #31168, #2285, #75179, #75638, #60515, #39162, #18342, #82731, #46735, #60054, #90290, #40098, #45807, #3199, #2744, #54319, #10761, #38238, #16943, #88892, #39619, #90742, #24041, #82274, #74716, #17883, #9836, #47197, #3682, #25900, #4145, #32083, #32567, #61459, #52916, #60984, #83194, #89832, #24993, #33016, #24507, #25442, #61907, #54782, #31624, #83661, #18825, #81795, #38709, #89351, #53389, #17426, #46275, #41017, #12660, #55741, #63803, #6017, #69940, #78456, #12174, #77511, #4602, #48141, #26853, #41973, #40556, #77043, #42444, #92632, #64285, #5083, #33964, #84593, #93113, #34430, #62868, #6485, #35364, #20221, #19743, #85069, #33475, #69470, #62378, #21147, #91223, #26390, #76581, #27804, #92167, #41505, #56697, #85543, #55278, #20691, #85998, #56210, #19282, #28268, #91701, #84132, #77997, #49561, #48611, #11704, #70433, #49099, #13592, #13137, #70887, #34892, #5559, #57157, #63336, #27324, #71354, #35826, #50956, #50017, #29184, #65666, #22086, #79839, #30116, #58543, #50493, #22535, #86452, #66569, #58081, #73216, #36744, #22997, #36281, #93567, #8783, #51407, #78910, #14979, #44772, #79394, #64740, #14057, #14530, #43835, #58999, #59470, #72737, #87388, #780, #44305, #30573, #15917, #7857, #29663, #73672, #37661, #80299, #15439, #43385, #51872, #87848, #86934, #80765, #8332, #6953, #42921, #37213, #66120, #1691, #1234, #88325, #71835, #28724, #57609, #21610, #72280, #7400, #65201, #304, #52346, #84361, #19056, #52803, #12410, #63104, #55036, #2637, #11940, #81681, #16830, #45687, #74595, #9724, #38603, #67507, #40789, #69242, #53272, #91471, #26622, #31516, #60404, #89242, #24395, #82156, #17312, #47441, #76350, #11476, #11648, #80941, #52059, #37833, #89413, #40495, #24567, #2801, #82336, #17005, #40962, #23649, #52515, #31684, #8953, #24101, #23176, #2352, #38771, #88954, #52982, #4544, #60578, #81391, #53455, #59659, #69884, #31229, #47622, #9897, #91161, #9418, #66739, #76988, #18764, #16086, #81855, #19225, #16539, #1865, #44938, #45394, #45874, #33419, #33904, #74780, #76525, #67675, #69413, #5023, #84075, #62321, #26326, #48083, #12117, #55221, #62811, #74294, #73839, #30757, #60115, #88502, #38305, #67220, #55686, #42387, #85491, #28673, #13539, #49964, #19684, #71299, #57558, #84537, #5962, #86403, #77454, #92112, #91646, #21557, #57103, #78855, #21094, #85008, #93515, #27266, #92575, #48553, #63279, #41917, #85943, #12598, #56153, #50441, #14005, #79344, #20162, #49042, #70830, #14479, #49508, #56641, #77937, #42865, #93059, #26800, #5501, #41444, #64229, #43337, #36230, #34836, #34374, #6427, #13081, #35776, #28215, #72234, #64689, #63747, #35303, #71779, #70376, #20638, #6901, #27745, #78398, #7348, #36692, #8281, #29612, #58490, #43786, #22945, #73158, #65148, #87796, #37161, #87335, #1182, #8732, #72686, #22483, #726, #65614, #51357, #80247, #7805, #66070, #30063, #37608, #15861, #44248, #44720, #15384, #249, #58948, #73620, #29132, #51818, #58028, #80711, #86882, #22036, #79789, #50905, #14931, #89873, #40139, #91265, #26429, #40598, #53905, #11745, #69512, #48182, #83236, #90329, #5126, #18383, #76152, #60558, #25034, #61947, #68586, #83703, #18865, #10336, #89396, #47722, #61027, #39664, #32131, #55322, #82773, #33058, #4184, #54825, #10802, #17925, #84172, #24550, #75677, #17468, #76622, #25944, #53434, #11285, #33518, #25483, #82318, #46318, #61497, #46776, #62424, #19320, #75222, #39203, #32608, #90784, #3722, #54362, #4643, #69055, #77083, #68115, #12214, #41060, #3241, #69986, #47240, #79433, #28305, #35865, #20262, #26894, #49138, #85581, #63377, #13632, #64782, #93607, #14102, #27363, #78952, #42966, #21659, #56735, #63844, #72320, #20728, #49598, #34003, #92207, #35405, #42010, #57195, #86036, #77556, #62907, #21185, #34471, #13175, #5597, #28765, #56252, #6529, #71396, #50056, #78035, #85112, #57648, #91743, #70926, #84635, #71871, #93151, #55782, #78494, #6993, #92676, #19784, #48655, #34929, #6057, #86496, #50535, #12705, #41545, #27846, #64325, #42483, #14569, #43425, #70469, #44807, #58125, #88364, #38160, #43876, #66153, #65707, #52383, #8818, #36323, #15017, #29230, #73708, #88820, #45727, #80332, #72773, #15951, #7898, #45257, #37698, #23968, #74161, #73256, #80803, #59515, #65237, #1269, #81260, #37249, #59034, #2209, #22570, #66604, #8368, #30151, #819, #9277, #1726, #343, #16405, #30613, #87881, #23514, #52842, #29700, #23033, #15475, #58583, #51912, #51444, #87422, #67075, #31093, #16868, #59981, #81719, #7441, #36787, #86970, #22124, #50992, #79877, #44346, #75106, #53789, #46201, #40476, #10216, #47121, #18267, #68940, #24912, #67998, #4526, #38639, #89752, #31550, #4071, #40024, #67542, #25366, #47604, #39543, #19206, #74637, #75563, #39084, #76507, #69393, #2671, #60442, #46659, #76034, #32006, #10685, #83583, #54246, #11163, #89278, #61833, #11630, #17350, #68465, #3126, #25826, #32941, #9764, #82196, #24429, #90666, #62301, #53311, #82657, #60904, #83116, #17806, #18746, #54706, #91141, #33402, #3600, #26308, #55203, #32487, #61384, #84058, #90217, #5946, #42847, #63262, #78381, #49026, #20143, #12580, #49947, #20621, #76969, #28198, #85474, #77922, #71282, #93500, #41427, #13064, #27249, #5484, #41900, #92093, #70359, #13522, #35284, #86388, #71763, #27727, #6886, #48535, #48065, #70814, #35760, #28655, #77436, #12098, #42370, #78840, #34357, #40944, #56135, #34818, #84988, #56624, #13986, #64673, #57086, #63731, #93041, #85926, #69865, #92556, #49492, #5003, #6409, #64212, #33886, #21076, #62794, #91629, #26782, #55669, #84520, #19667, #29595, #44702, #73603, #65133, #21539, #8714, #22020, #710, #86866, #81156, #50890, #87779, #58929, #15845, #65597, #14914, #45153, #79327, #36675, #72217, #37591, #80691, #14464, #66052, #88253, #80232, #59875, #50422 ),
 ( #58474, #38049, #73139, #79771, #74052, #9171, #22929, #87318, #30048, #43321, #7333, #36213, #234, #29114, #58010, #43769, #66502, #37145, #51338, #1621, #30504, #72670, #59399, #30988, #1165, #7790, #66958, #22466, #15368, #51799, #23411, #44230, #8265, #52277, #16300, #2097, #90112, #68356, #54141, #82556, #11524, #89171, #24323, #3484, #74516, #89633, #88715, #67894, #10577, #60795, #24803, #68834, #32377, #53200, #61278, #31445, #40371, #3017, #18162, #75456, #61726, #75003, #38536, #47493, #25264, #23863, #53689, #83471, #82078, #9651, #52729, #17236, #17704, #3962, #4417, #18627, #76402, #83010, #31903, #47015, #16761, #81612, #45615, #33295, #67439, #2566, #60334, #75918, #39440, #46557, #11043, #32836, #46098, #39913, #10115, #90558, #38981, #69288, #25716, #54600, #63623, #49385, #26192, #91023, #76863, #34709, #78277, #92448, #41795, #27611, #56022, #78732, #62684, #91517, #70706, #47959, #63153, #62193, #41310, #77807, #34247, #91984, #42259, #5837, #26673, #56508, #4887, #13875, #70247, #85367, #48905, #35170, #48425, #11988, #20968, #20517, #55086, #27137, #56979, #55563, #40837, #83955, #84411, #84877, #71173, #71643, #20028, #13415, #12957, #6302, #42728, #28093, #64092, #92932, #85817, #49835, #6776, #19104, #19559, #69756, #33771, #5382, #77330, #12463, #86277, #93393, #80117, #29480, #66389, #51229, #87665, #57436, #15256, #1505, #28545, #43663, #30391, #21430, #36104, #35653, #59283, #1056, #22815, #58820, #29005, #37479, #65022, #36565, #50304, #7229, #79667, #29935, #79209, #122, #88129, #51684, #23287, #57890, #86746, #14808, #52160, #87207, #21908, #81043, #73020, #72558, #44117, #14352, #43212, #72113, #73939, #50782, #7680, #64568, #80573, #8148, #65480, #15726, #44587, #597, #73491, #45037, #37031, #58366, #16186, #22355, #65945, #8602, #89996, #66841, #37932, #23750, #75342, #25151, #10458, #82442, #68242, #2903, #25603, #9528, #38413, #17590, #88602, #9998, #9054, #81960, #24684, #74887, #38870, #82891, #46439, #67322, #39324, #45496, #54486, #17117, #32254, #89520, #75801, #89056, #52613, #61614, #3365, #1976, #67776, #3845, #2454, #81495, #30867, #31330, #31786, #18048, #18505, #60680, #61160, #53567, #54025, #83355, #68715, #46900, #10925, #32727, #90446, #39793, #47368, #60217, #59761, #16642, #45982, #74398, #24205, #53082, #40260, #27022, #70129, #13303, #91868, #34599, #4305, #55911, #42141, #69176, #84297, #71059, #62072, #76745, #76282, #6191, #41679, #63509, #5724, #69641, #78165, #11873, #77214, #33183, #47843, #26557, #70597, #90906, #40725, #35058, #92337, #63978, #4769, #33652, #55445, #92818, #34134, #62561, #27981, #26073, #54961, #48313, #48784, #91402, #12342, #85252, #84763, #19913, #83837, #27492, #56871, #18991, #41190, #19447, #56390, #77691, #11408, #5265, #63037, #12841, #85713, #20858, #20399, #49270, #58264, #57330, #87559, #22257, #66288, #22705, #21804, #29373, #8037, #78626, #14706, #954, #79563, #7574, #44486, #64917, #80013, #50677, #43559, #14246, #51579, #51130, #13768, #29832, #87107, #72455, #72911, #1401, #43104, #36459, #28898, #7128, #65374, #20, #72011, #15153, #36932, #59175, #73390, #44013, #8500, #50193, #49729, #486, #37378, #30288, #79097, #88020, #65846, #80465, #35998, #42617, #57786, #58715, #86636, #15614, #71536, #6669, #35546, #64459, #93285, #28437, #86172, #21323, #87811, #2600, #15880, #73638, #58045, #22500, #59437, #66085, #81188, #16335, #7819, #86896, #45184, #58506, #37178, #29627, #23896, #87351, #30535, #1656, #52311, #8296, #51372, #81646, #22051, #73177, #14945, #74087, #23443, #50920, #8748, #31021, #22960, #79804, #43800, #58964, #80263, #59908, #52766, #88750, #72700, #1198, #16794, #36709, #15399, #65630, #45648, #9206, #38084, #66995, #44266, #74558, #30079, #51834, #743, #80727, #44736, #2132, #37626, #66536, #9687, #38569, #67471, #88288, #62098, #76769, #49291, #84317, #3052, #56413, #85273, #70151, #11897, #41214, #53234, #89207, #82117, #71081, #17275, #24358, #31480, #19936, #48335, #62583, #48806, #41702, #46132, #77713, #42166, #12366, #67928, #78186, #54985, #75035, #34157, #12863, #10148, #60368, #39014, #5287, #70619, #63060, #91889, #27043, #26579, #13324, #31937, #90931, #55931, #26096, #33674, #83861, #40746, #77236, #4795, #91425, #5746, #84786, #19014, #34621, #47866, #69663, #55468, #63531, #19468, #92358, #27520, #20422, #58739, #72479, #35082, #64940, #974, #6693, #20880, #64001, #35568, #7148, #15176, #15637, #72033, #43581, #21824, #511, #80489, #65866, #36023, #50699, #29855, #87582, #41, #79587, #64482, #72936, #44034, #79121, #36953, #14728, #56895, #92839, #7595, #28921, #22727, #36481, #58285, #28002, #65398, #87128, #44506, #51601, #29393, #6213, #93309, #85734, #57809, #49752, #78649, #28459, #13789, #22279, #8062, #86194, #42641, #21346, #86660, #57353, #51151, #71558, #50217, #80035, #14268, #43128, #24594, #61073, #2374, #9444, #17963, #31252, #88978, #73412, #37858, #74805, #81414, #2826, #31709, #23202, #8522, #60601, #73861, #52539, #44961, #39243, #8979, #45900, #17034, #67698, #23673, #66762, #3279, #37401, #88525, #30310, #89436, #38794, #66311, #24126, #46360, #38331, #1426, #59199, #74319, #1893, #75261, #68159, #88046, #52082, #45419, #9921, #30784, #67244, #82359, #53005, #53483, #80965, #17508, #10376, #16110, #60139, #59682, #32172, #89915, #16564, #81879, #25071, #53944, #82812, #85159, #25983, #54402, #55360, #83275, #84678, #19359, #63421, #19827, #18905, #26471, #5172, #75718, #11785, #91783, #76658, #4683, #41590, #61988, #77125, #47760, #40635, #11325, #48694, #48223, #10841, #26934, #84212, #69554, #70029, #92250, #40176, #33557, #54868, #4222, #62467, #90823, #69095, #12255, #70512, #47279, #46816, #91309, #5639, #27407, #76196, #56295, #41100, #77599, #33098, #39705, #83749, #34046, #62949, #55822, #12749, #34514, #68629, #3762, #32647, #61535, #90367, #25523, #18419, #58626, #71919, #35910, #20312, #78538, #21709, #28350, #43471, #72368, #63887, #49182, #7485, #20771, #93198, #85625, #79923, #49643, #86539, #57696, #14614, #64372, #13677, #43922, #78076, #35454, #70969, #36370, #79479, #13219, #64828, #87016, #78997, #42055, #6102, #21233, #42528, #22168, #15060, #34973, #92723, #86082, #50585, #71439, #50102, #29277, #93652, #65283, #27894, #388, #51036, #56783, #14151, #6576, #58174, #72817, #57240, #43016, #7040, #7943, #36838, #28812, #65756, #866, #29745, #1314, #31599, #60029, #10265, #60488, #59563, #67124, #45776, #22614, #52431, #38684, #23563, #45304, #82245, #8865, #24015, #88413, #81306, #51959, #89325, #88866, #51489, #67589, #31142, #16452, #16918, #39135, #80851, #74209, #66651, #44850, #9327, #37743, #15998, #52888, #74687, #3173, #17401, #2260, #46249, #81768, #75153, #87928, #87467, #38210, #68046, #32057, #23079, #80377, #9811, #24480, #73753, #15518, #1777, #2719, #30661, #53359, #44393, #73302, #8413, #37292, #66198, #30196, #59086, #83631, #90712, #5532, #18794, #76554, #60951, #25415, #62351, #68988, #84107, #19256, #10735, #89802, #48114, #61433, #40071, #32541, #26828, #90265, #33449, #4575, #55251, #11213, #54293, #84566, #24965, #76081, #17857, #77018, #26360 ),
 ( #12146, #91192, #53840, #68514, #82706, #40991, #48584, #46708, #4118, #3650, #69444, #83165, #5052, #69914, #77484, #33935, #32990, #40527, #62843, #75611, #25872, #91676, #54754, #47653, #55715, #61881, #19713, #11677, #12628, #18316, #41474, #70406, #39592, #47172, #71807, #64259, #57586, #79818, #92605, #93089, #13566, #85519, #28243, #49535, #27775, #64715, #21589, #43814, #34402, #50468, #34863, #42416, #5991, #283, #63776, #6929, #35802, #28701, #78429, #56669, #58059, #92140, #71328, #85041, #86430, #93542, #27295, #78885, #7377, #57130, #72714, #63309, #35333, #20664, #36258, #29163, #56182, #20190, #6458, #79371, #85972, #21122, #43364, #14032, #14508, #49070, #72260, #65178, #70859, #49990, #42893, #86911, #22066, #77968, #41947, #13110, #50934, #14959, #46146, #80743, #15416, #16348, #44284, #45665, #74101, #24372, #74573, #73652, #81202, #59925, #36724, #66548, #52782, #37640, #59450, #2616, #22977, #38101, #8762, #1669, #66100, #9701, #9220, #65643, #81660, #45198, #30552, #31035, #53251, #1212, #88301, #15894, #58977, #23458, #51850, #30094, #67011, #88764, #17289, #31494, #2146, #60382, #8310, #7837, #52325, #89221, #82133, #37193, #757, #23910, #38582, #87826, #29642, #44751, #16808, #67485, #58521, #87365, #22515, #51386, #80277, #73191, #26245, #62735, #4008, #11097, #19608, #32883, #90604, #75050, #39486, #76447, #83058, #4465, #33342, #24853, #67943, #91074, #84458, #54647, #17750, #26722, #3536, #89687, #11568, #62239, #39030, #10161, #53737, #47543, #55138, #40416, #83521, #69334, #68878, #91566, #75505, #10627, #18679, #60844, #75968, #3066, #54188, #25765, #47062, #39962, #84001, #19149, #68407, #48005, #46603, #55609, #18212, #76909, #61771, #12039, #61324, #82603, #33826, #40886, #31951, #69804, #4940, #32425, #90162, #25310, #48959, #49435, #57484, #57942, #20563, #85866, #64148, #42781, #29050, #14400, #78323, #92981, #43259, #72157, #13463, #28139, #13006, #21477, #86326, #27664, #79260, #57028, #5429, #12514, #21017, #42313, #7273, #49885, #6826, #70298, #78782, #36150, #41364, #56562, #65071, #34295, #77856, #48477, #170, #13923, #35700, #71698, #41842, #50355, #70754, #71222, #63202, #20079, #92495, #64614, #92032, #5887, #86797, #93440, #77376, #34757, #63672, #85415, #27187, #6349, #35222, #56074, #84927, #28594, #1099, #30435, #43707, #79712, #72606, #60263, #7728, #14854, #21955, #9100, #37522, #51727, #37977, #30916, #22862, #87711, #80166, #23794, #88178, #50828, #2024, #59327, #80620, #45082, #67367, #15304, #15776, #29980, #73069, #44634, #37079, #44163, #52206, #66885, #31374, #16686, #1552, #45541, #22401, #36609, #73536, #74442, #2496, #51273, #65529, #16232, #52658, #8200, #646, #65988, #8645, #58864, #23338, #81538, #9574, #59805, #66432, #88646, #38463, #29529, #81088, #73983, #58409, #87255, #10967, #89100, #53615, #90487, #3407, #18547, #47415, #38912, #24252, #76325, #89562, #68285, #60723, #55008, #24732, #61654, #32766, #83397, #39369, #82485, #19031, #53126, #10500, #46028, #11450, #54528, #82006, #39835, #62119, #54066, #33693, #17163, #90040, #17633, #90950, #83881, #74932, #10042, #61205, #25645, #46484, #25192, #4346, #68759, #40302, #67821, #69217, #26114, #31832, #82936, #75387, #33223, #47885, #2946, #32299, #18088, #76789, #11915, #46942, #75844, #3889, #40764, #69682, #4812, #35099, #79137, #6711, #34638, #42183, #20898, #91447, #27536, #13806, #92377, #20441, #57370, #77732, #92857, #91908, #71096, #93325, #28477, #42658, #55949, #71575, #35585, #50234, #85291, #56429, #7166, #49309, #78203, #62604, #27062, #64017, #70636, #85751, #49770, #12386, #26597, #78665, #63078, #41720, #34176, #86212, #84804, #28021, #6229, #56911, #12883, #19954, #21364, #55487, #5764, #19487, #64499, #14286, #84336, #13342, #43147, #72050, #48353, #77256, #63548, #48825, #41232, #70172, #5307, #59, #9345, #9828, #88432, #67143, #46266, #81786, #74707, #87946, #24498, #68065, #73771, #2277, #1796, #82264, #38701, #64958, #44868, #57826, #67608, #24983, #75629, #16469, #8884, #45797, #37763, #75170, #2736, #53856, #10283, #38231, #16935, #89342, #28940, #31160, #17417, #60046, #88884, #32074, #52448, #31616, #24032, #52908, #30681, #39153, #60507, #23098, #3190, #53379, #60973, #89822, #82722, #59581, #17874, #45324, #23581, #46726, #81322, #74226, #36041, #51980, #80869, #16016, #66668, #5550, #11234, #10752, #11695, #63327, #56201, #40089, #85060, #5073, #12649, #90732, #3671, #25891, #62369, #32558, #77034, #92158, #49089, #83650, #18332, #19273, #47188, #48602, #12165, #27315, #77502, #76572, #84123, #62859, #39609, #69461, #55732, #40546, #91212, #34420, #54773, #41008, #4593, #33466, #69005, #41494, #69931, #68533, #84584, #48131, #26380, #33955, #20211, #4136, #55268, #18814, #61898, #91692, #47671, #33007, #26844, #19734, #61450, #90281, #70424, #25432, #54310, #83185, #76101, #36737, #29656, #13583, #58536, #72273, #79832, #64276, #70877, #93105, #35818, #42435, #57602, #14972, #43828, #58073, #71345, #29177, #86926, #65658, #6945, #14049, #22528, #64732, #93559, #77987, #6476, #79386, #85989, #7392, #36273, #27794, #13128, #65194, #78447, #57148, #49552, #72729, #35354, #50484, #21603, #297, #28260, #21139, #7850, #41964, #50009, #34883, #22079, #43378, #6008, #28717, #50949, #42912, #63794, #92623, #78902, #71826, #772, #87381, #56687, #85534, #86445, #14523, #20681, #81216, #60397, #2160, #88778, #8324, #38596, #82149, #87840, #16362, #15909, #2630, #52796, #80291, #58991, #67499, #74588, #44765, #53266, #80757, #52338, #73205, #22990, #1684, #16824, #15430, #51864, #17304, #31509, #39045, #73665, #8776, #30565, #67956, #9235, #37654, #75064, #10175, #23926, #59463, #59939, #37206, #44297, #66114, #89702, #1227, #30109, #51400, #89235, #67024, #45213, #24388, #46161, #66562, #3081, #60859, #31049, #88315, #31966, #23472, #74115, #81675, #38114, #45681, #9716, #39501, #91089, #12054, #26260, #4480, #84016, #18695, #41379, #25325, #54205, #33357, #10641, #25781, #24869, #4026, #40432, #90619, #54663, #4955, #62255, #83073, #55154, #61342, #70313, #32899, #48021, #11585, #91582, #11112, #68422, #77392, #19164, #53751, #83536, #19624, #18227, #3552, #82617, #47078, #47558, #33841, #34311, #76463, #76926, #69350, #40901, #5444, #84474, #69821, #62750, #48492, #12529, #26739, #55625, #75984, #63217, #17764, #61787, #46618, #75519, #32441, #90177, #39979, #68894, #50372, #28154, #6841, #84944, #85881, #79276, #27203, #78338, #14417, #48976, #5903, #92049, #43274, #71714, #72172, #13021, #63688, #56090, #7288, #35715, #57499, #28610, #20578, #36166, #56577, #64164, #41857, #27679, #42327, #64629, #77872, #85430, #65087, #86343, #187, #49450, #13480, #71238, #20094, #93455, #6367, #70770, #34773, #92513, #21494, #35238, #21033, #57043, #49901, #92996, #78796, #13941, #42798, #70139, #4780, #19001, #5276, #91879, #75813, #34145, #92347, #62571, #25615, #34610, #11419, #3856, #84306, #63049, #46912, #18059, #32736, #55455, #27033, #19458, #91413, #48323, #76757, #5735, #83367, #18517, #26567, #68726, #83849, #82905, #62085, #33661, #54973, #47854, #55922, #77225, #47381, #12353, #54497, #63520, #90918, #41202 ),
 ( #76294, #48794, #40271, #84774, #19923, #77703, #33194, #69187, #12852, #10937, #4317, #39804, #41690, #70608, #61625, #27502, #90458, #11884, #26084, #40734, #69651, #36011, #14717, #85262, #21335, #7584, #86184, #14257, #51141, #71546, #86647, #57343, #28448, #20869, #58275, #28910, #20411, #36470, #30, #50204, #79574, #8049, #49741, #79108, #35557, #13778, #43115, #6680, #78638, #21813, #43570, #65855, #80025, #64929, #15165, #56883, #56401, #72021, #44023, #36942, #85723, #963, #50688, #87116, #42627, #49280, #64470, #7138, #93298, #57797, #22266, #72921, #65385, #72468, #498, #29381, #78176, #13314, #42153, #71070, #6202, #35068, #63988, #92828, #27991, #37843, #52992, #81866, #73399, #29842, #17015, #30298, #8965, #1411, #89423, #59185, #2361, #67231, #24112, #73848, #23187, #53466, #87570, #44948, #80474, #45884, #88965, #22714, #74304, #2813, #88512, #68147, #58725, #30769, #88029, #31695, #24577, #51589, #15624, #1875, #31239, #80952, #59669, #38781, #9428, #60126, #8509, #74791, #60588, #52069, #23660, #66749, #9908, #67685, #37388, #52526, #81401, #82346, #17494, #16550, #45405, #38316, #46347, #75248, #10363, #39230, #19813, #41087, #69080, #61522, #5156, #62935, #25059, #61059, #4208, #69537, #54388, #33083, #12240, #47746, #40621, #53931, #84198, #34032, #39689, #61974, #90353, #48207, #4670, #32157, #10829, #82800, #33543, #84661, #41576, #76181, #68615, #11769, #3750, #70012, #62449, #48680, #91769, #90809, #76644, #55346, #89901, #25968, #77110, #54850, #83733, #26921, #18407, #91294, #18891, #26457, #25510, #55808, #19345, #17951, #77582, #12733, #3267, #46803, #75706, #83262, #32632, #11312, #47265, #40163, #85612, #34960, #7027, #57683, #79910, #65269, #50088, #374, #70955, #70498, #71426, #29261, #22154, #6087, #51022, #64815, #72354, #56770, #63407, #20758, #28337, #63872, #78983, #7471, #36355, #50569, #92707, #21691, #79465, #58157, #93185, #6559, #15047, #57227, #86069, #5625, #27879, #71906, #78525, #93639, #28798, #20297, #34500, #86526, #49630, #13663, #42040, #87002, #42515, #43002, #14136, #14599, #35439, #64360, #92236, #27391, #21219, #56281, #43457, #35897, #85142, #49169, #78062, #13205, #82230, #43908, #44837, #38196, #45763, #30183, #36820, #59071, #1764, #73288, #23549, #74673, #9797, #24002, #37278, #88853, #52875, #31586, #66637, #73740, #72804, #30648, #59548, #7929, #8400, #45291, #51944, #67109, #2244, #87454, #65742, #31128, #44378, #23066, #15505, #38671, #66184, #16439, #81293, #60014, #87915, #1301, #67576, #851, #80836, #29732, #81754, #9313, #58613, #88399, #16905, #8852, #22601, #51476, #37730, #15985, #2704, #60475, #80364, #52418, #74195, #89311, #24466, #53346, #26344, #61866, #54739, #68032, #4560, #48100, #53826, #76066, #75596, #62338, #18778, #46236, #24949, #39120, #83617, #5039, #55701, #90250, #82692, #25857, #17842, #55237, #47637, #33919, #84093, #83148, #90697, #69430, #75140, #11196, #91178, #47157, #68973, #12133, #32524, #76540, #18299, #40056, #10719, #19242, #11663, #10251, #77004, #40511, #4103, #33434, #62828, #39576, #32974, #25398, #68499, #40978, #61418, #3633, #69900, #91662, #26816, #17387, #3159, #32043, #46694, #60937, #89785, #54278, #36244, #20177, #65162, #41934, #78415, #5979, #49057, #21109, #71793, #265, #79358, #64245, #14493, #85026, #84553, #85506, #43351, #29148, #77953, #19700, #78870, #86416, #70845, #77471, #34851, #42404, #13096, #93075, #21573, #50455, #64702, #63763, #35789, #93528, #72247, #13554, #20653, #48569, #71314, #6445, #12614, #92593, #85957, #27762, #14019, #42880, #34389, #41459, #6915, #56657, #49523, #56169, #7362, #35320, #57117, #28229, #28687, #49977, #57573, #70391, #5519, #63295, #92127, #27282, #28277, #26863, #13602, #35835, #27816, #7410, #62877, #63812, #27334, #64751, #28736, #84605, #55751, #34901, #35376, #20232, #92644, #71842, #42453, #6495, #19754, #50026, #93577, #5569, #56706, #56221, #14068, #64295, #91711, #70442, #48621, #93121, #50505, #77522, #41982, #34440, #71365, #63346, #6962, #57167, #79403, #57619, #20700, #86007, #21157, #12674, #49570, #42933, #78465, #78919, #86462, #78006, #21623, #14539, #43394, #85081, #72288, #41516, #92179, #49109, #13146, #70895, #6027, #82975, #789, #67406, #16724, #24771, #46524, #29196, #53653, #46982, #17203, #72745, #18128, #58552, #50965, #38950, #82523, #313, #65209, #79848, #10082, #17671, #67861, #46064, #2985, #31413, #54103, #36755, #65677, #74969, #22095, #38501, #36291, #45578, #53165, #9614, #2534, #75425, #31871, #29671, #60759, #7866, #75882, #74483, #89601, #24289, #10543, #22543, #14988, #90078, #39408, #58093, #60301, #32343, #87396, #43847, #86943, #51417, #89139, #68324, #81575, #82046, #3447, #61243, #25230, #85329, #70670, #40802, #55525, #5799, #34672, #11953, #84375, #69255, #77771, #19989, #83918, #41759, #19523, #61691, #68797, #48390, #4850, #63588, #26636, #63118, #32802, #77293, #92412, #3926, #19069, #27572, #90522, #11490, #11008, #56470, #70212, #91945, #34212, #4383, #12919, #40339, #69719, #25684, #76363, #55049, #5346, #54565, #33261, #20479, #27100, #49346, #62158, #90987, #47925, #39876, #62647, #26157, #83434, #18589, #12423, #76827, #41275, #47456, #33735, #91484, #55986, #84840, #48867, #22783, #65446, #93, #14319, #1027, #22326, #50264, #57857, #36531, #13378, #43179, #29446, #72081, #36072, #72986, #93358, #14776, #79174, #7197, #42692, #80084, #50750, #42220, #58335, #21878, #64989, #7646, #29905, #71611, #28972, #57402, #35618, #86712, #28509, #6745, #43629, #562, #87633, #8116, #79634, #37002, #78699, #78241, #72526, #65914, #58789, #13840, #71134, #87177, #15227, #64533, #6264, #86243, #51197, #21394, #44083, #35132, #64055, #92897, #28056, #56946, #85783, #20934, #49802, #81465, #89968, #9493, #67293, #51652, #16157, #53054, #59732, #74857, #9969, #1474, #80538, #38841, #52133, #30837, #23255, #17559, #81013, #24173, #89026, #45951, #1940, #45008, #75311, #15695, #66810, #8571, #67748, #17082, #44557, #2422, #24649, #16614, #73460, #37450, #52585, #73910, #53538, #46411, #66359, #30360, #23722, #81929, #9026, #45469, #60650, #31302, #2874, #59249, #31758, #82412, #88095, #74369, #37905, #89488, #10430, #88574, #38381, #60188, #39294, #68213, #3332, #32222, #61131, #33616, #32698, #63006, #91366, #53996, #61584, #46870, #26525, #12808, #63474, #4273, #90416, #62524, #25573, #91836, #55413, #41649, #26991, #90875, #4737, #77181, #82865, #83804, #70089, #54923, #76712, #19881, #40230, #84266, #26039, #18957, #83326, #55880, #19416, #18017, #5232, #48279, #47811, #12311, #70566, #18472, #11838, #33151, #76249, #40689, #69145, #47332, #41155, #34104, #34565, #48752, #84732, #77657, #54453, #25122, #69607, #5691, #75774, #11379, #10894, #39758, #68685, #62041, #3817, #78591, #50160, #27948, #71974, #29333, #58228, #72424, #85678, #43527, #7540, #79979, #21287, #28404, #36892, #79058, #14209, #92303, #56838, #93709, #6630, #21767, #50643, #42108, #27460, #79532, #92779, #71498, #63941, #87072, #20826, #64883, #35964, #86597, #42583, #49695, #22220, #56352, #13731, #49237, #14671, #57752, #85214, #43070, #65342, #57296, #20367, #78133, #93251, #35510 ),
 ( #449, #51090, #13271, #71023, #64425, #28864, #86138, #7093, #36425, #15116, #43975, #6155, #72876, #8000, #35027, #30718, #30249, #16969, #67178, #919, #73353, #87524, #38266, #53414, #10317, #44902, #8465, #74259, #37345, #9860, #2311, #82298, #38734, #37796, #45357, #24067, #29798, #59616, #45835, #1832, #23614, #60538, #80904, #31195, #66703, #88467, #59140, #67640, #60080, #58678, #74740, #9383, #52481, #88917, #17449, #87983, #81355, #73805, #23135, #16505, #16050, #52018, #52943, #81820, #75202, #89376, #2766, #24532, #66251, #65808, #31648, #46298, #22670, #1366, #51542, #80431, #15577, #8919, #44447, #25463, #90765, #68568, #18846, #69966, #5107, #19302, #32589, #84154, #48162, #26876, #61928, #69036, #77535, #25924, #54807, #39185, #3704, #40579, #47223, #62405, #91247, #82753, #68097, #26411, #39644, #18363, #10783, #33985, #61480, #11726, #76603, #33497, #83218, #90311, #62888, #3222, #54343, #89854, #55301, #4624, #32112, #83685, #12196, #41038, #4166, #61009, #25015, #40120, #76133, #91724, #55763, #53887, #17905, #11267, #69494, #33039, #47704, #77065, #84616, #19765, #46759, #48634, #75659, #49119, #71375, #70905, #57630, #14082, #41526, #20242, #34450, #78931, #324, #50976, #85562, #78016, #21167, #13156, #50517, #42946, #29209, #79415, #78475, #86017, #64763, #70452, #6508, #86473, #42465, #64307, #7421, #27828, #71853, #13612, #35387, #6039, #14550, #6974, #5579, #21639, #50036, #93131, #35846, #58108, #34911, #28286, #20710, #63822, #57177, #56716, #92656, #93588, #28747, #22106, #36303, #43407, #65219, #41992, #12685, #72301, #86954, #63358, #49580, #92189, #27344, #56231, #85094, #72756, #66138, #37680, #15456, #59495, #16848, #45704, #59962, #73239, #31074, #88801, #67523, #8801, #15936, #24410, #66588, #1709, #79861, #44328, #81241, #87866, #9261, #38138, #29682, #14999, #67054, #80316, #59019, #51427, #74617, #8350, #52366, #23498, #74143, #30135, #37233, #9745, #43858, #1253, #36768, #2189, #45238, #7877, #30592, #65688, #802, #58565, #87406, #22553, #23015, #51894, #23948, #88347, #44790, #52820, #81700, #80787, #38619, #89259, #16388, #73691, #31532, #2653, #60419, #54688, #40457, #17332, #82176, #67979, #25808, #69375, #83562, #32923, #18723, #47103, #69849, #53773, #82639, #61813, #39066, #54228, #53289, #32467, #68921, #25347, #83096, #33384, #90646, #17789, #47585, #89730, #4983, #61366, #76489, #40005, #26289, #39523, #3105, #12080, #11612, #46182, #18250, #48048, #46642, #31988, #75087, #75543, #76010, #62283, #62778, #11142, #4505, #4053, #91119, #33868, #19189, #55184, #84043, #76953, #40928, #91611, #10197, #10668, #60880, #24893, #90199, #68444, #3578, #77419, #84504, #71268, #20607, #57530, #42355, #78827, #48519, #6396, #86375, #19650, #34801, #21526, #12559, #27231, #26766, #50405, #85911, #13972, #49930, #20123, #28641, #56120, #27709, #41409, #92077, #70796, #21063, #70343, #84973, #79311, #42831, #14451, #49008, #77905, #5931, #43308, #78368, #13048, #72203, #7321, #64196, #63716, #35268, #41885, #36199, #92541, #93027, #28184, #71747, #56606, #85460, #65118, #5469, #49477, #34339, #6874, #35746, #63246, #57073, #93488, #13507, #55651, #64660, #1152, #58461, #2082, #59860, #22007, #57995, #66039, #66490, #51324, #30035, #9155, #44689, #37579, #50877, #81142, #30971, #36663, #58916, #87305, #45137, #1605, #29101, #7777, #79759, #30490, #81596, #38520, #73124, #65583, #8699, #697, #38035, #59385, #16746, #66942, #87762, #73590, #52262, #86849, #22916, #74038, #51786, #80676, #88701, #15356, #88237, #15831, #23395, #22452, #23849, #16286, #14900, #52715, #45601, #74503, #9633, #221, #80217, #43756, #8250, #44216, #72655, #37132, #29581, #3949, #54585, #76846, #62177, #47001, #91009, #67880, #67425, #68343, #26178, #19090, #3003, #47944, #61711, #69274, #53672, #60321, #82540, #25249, #31889, #75904, #4403, #33282, #47476, #60780, #18612, #76383, #55068, #90098, #3470, #11973, #54125, #82996, #2553, #89620, #68818, #75443, #90545, #25703, #17221, #31432, #83457, #24788, #46541, #83937, #32362, #18147, #89159, #24308, #61262, #11029, #17691, #40357, #11510, #10562, #53187, #39897, #82065, #46082, #32821, #74990, #10101, #38968, #39426, #62667, #21783, #72889, #4872, #50176, #8013, #26656, #42597, #40821, #36907, #7555, #29351, #65355, #35526, #43992, #71512, #43085, #91500, #13749, #86152, #36440, #33755, #6646, #65825, #58243, #29811, #64439, #93265, #21303, #58692, #3862, #28419, #932, #87536, #79545, #79072, #50659, #55545, #84395, #19544, #80444, #48410, #77313, #69740, #87086, #57767, #71989, #22235, #51106, #57310, #79992, #51556, #14685, #14224, #22683, #7107, #35978, #43540, #15129, #64898, #28879, #86613, #72437, #462, #2330, #9397, #31209, #52494, #24546, #23151, #52035, #38281, #66265, #59635, #15589, #1846, #74274, #88482, #23629, #45850, #67194, #80921, #60094, #16064, #53430, #30733, #24082, #45371, #38751, #8933, #59154, #89392, #88933, #73367, #81371, #31662, #44918, #1380, #8479, #73820, #16520, #74756, #17464, #52958, #81835, #16985, #9875, #44462, #67655, #2781, #30262, #87998, #37811, #37358, #60554, #82314, #66718, #87380, #22078, #36272, #22527, #15429, #93103, #51399, #15908, #79831, #42910, #51863, #28715, #21137, #7849, #80290, #64274, #35352, #50007, #72728, #44296, #36736, #14971, #65657, #296, #22989, #6943, #35816, #43827, #85987, #7391, #6474, #79385, #50948, #72272, #65193, #73204, #771, #64730, #29655, #71824, #80756, #14522, #58535, #86925, #8323, #86443, #78900, #58990, #37205, #28258, #29176, #1226, #93557, #14047, #57146, #57600, #58072, #66113, #44764, #30108, #87839, #21602, #50483, #43377, #39500, #9715, #24387, #68421, #3551, #74587, #53265, #38113, #46617, #82616, #52795, #10640, #82148, #30564, #37653, #17303, #67498, #32440, #89234, #31965, #1683, #46160, #61341, #66561, #81674, #90176, #59462, #74114, #73664, #25324, #39044, #60858, #3080, #67023, #75518, #9234, #38595, #88314, #45212, #23925, #67955, #23471, #2159, #54204, #89701, #83072, #31048, #59938, #16823, #18226, #31508, #88777, #8775, #52337, #75063, #45680, #10174, #24868, #81215, #16361, #53750, #2629, #60396, #17763, #48020, #5902, #92512, #76462, #27678, #41378, #48975, #33356, #39978, #62254, #4954, #11584, #26738, #77871, #13020, #27202, #40431, #92048, #56089, #34772, #69820, #76925, #85429, #33840, #62749, #47077, #69349, #48491, #55153, #70312, #5443, #90618, #75983, #34310, #47557, #26259, #18694, #41856, #4479, #19623, #84473, #63216, #91088, #84015, #70769, #11111, #19163, #4025, #84943, #12528, #68893, #91581, #20093, #12053, #32898, #61786, #40900, #55624, #63687, #56576, #25780, #54662, #77391, #83535, #71713, #50371, #29547, #65086, #57960, #71237, #7744, #51291, #57042, #79275, #78795, #65549, #21972, #49449, #28153, #42326, #86814, #8218, #58883, #93454, #85880, #29068, #21032, #58427, #50845, #37096, #87273, #86342, #186, #72622, #78337, #14416, #663, #43273, #72171, #15321, #35714, #79728, #21493, #7287, #13940, #22419, #14870, #13479, #80183, #43724, #36165, #36627, #66005, #42797, #44182, #28609, #6840, #73088, #64628, #1117, #49900, #29998, #6366, #57498, #20577, #35237 ),
 ( #64163, #92995, #9119, #24271, #88664, #59823, #52224, #89582, #60283, #22881, #67841, #31393, #23813, #17184, #39390, #81107, #52676, #66905, #45100, #81557, #37996, #16250, #53146, #74952, #3427, #82505, #67386, #17653, #88198, #87729, #16705, #46504, #68305, #23357, #32323, #82026, #24753, #74002, #80640, #2044, #45560, #30933, #2516, #53635, #75407, #2967, #74462, #38932, #31852, #10523, #9595, #38482, #51748, #89120, #46047, #15795, #10062, #60741, #44654, #73555, #8664, #37542, #66453, #1570, #30453, #59347, #32785, #27081, #90505, #33714, #4830, #55507, #11470, #54547, #84821, #25212, #76344, #18110, #84356, #26616, #54085, #11934, #34194, #26135, #5780, #61225, #62138, #25666, #63098, #55968, #82955, #46962, #33243, #62626, #18569, #90969, #70652, #40783, #3908, #12901, #83415, #75864, #91465, #48373, #10987, #90059, #39857, #19505, #77275, #12404, #69701, #41252, #55030, #77750, #61673, #47435, #70193, #68779, #83899, #40321, #69236, #76809, #19050, #47906, #5326, #91926, #4365, #19970, #48845, #41739, #42673, #57839, #21377, #7628, #20915, #78221, #87159, #7179, #63568, #93340, #29425, #35114, #49327, #92394, #64034, #35599, #43612, #44066, #6727, #72062, #50247, #28953, #15209, #542, #64514, #79153, #58315, #22308, #28491, #14301, #92876, #36513, #72508, #13821, #65428, #43161, #85311, #27554, #36054, #57384, #51179, #64972, #86693, #56449, #75, #80066, #20459, #71590, #72967, #13360, #28038, #34654, #42201, #21858, #50732, #79616, #56927, #71115, #85765, #86227, #6245, #49784, #78681, #14758, #65895, #8553, #67731, #89009, #89470, #66342, #37433, #52114, #24631, #59714, #73443, #31740, #60633, #45452, #80997, #16596, #29887, #1007, #58771, #46394, #87613, #22763, #8096, #24156, #23705, #37888, #53036, #17064, #51634, #81912, #80520, #15673, #52568, #1923, #38824, #81448, #60171, #44540, #74352, #2858, #1456, #16139, #53518, #30342, #59232, #36983, #82394, #67275, #45931, #31285, #88078, #9952, #23234, #9009, #44991, #73892, #66793, #2405, #30817, #88557, #17542, #74839, #9475, #38361, #10877, #25557, #91821, #33135, #46853, #5215, #34087, #18939, #54437, #83785, #3315, #39277, #32204, #19866, #61111, #68195, #75294, #62507, #90859, #11360, #91347, #84249, #89950, #26507, #84717, #54906, #18000, #26974, #3800, #25105, #76696, #55397, #53979, #10413, #82848, #47794, #19400, #11822, #40673, #69591, #69129, #55865, #75756, #39740, #4721, #68664, #76230, #32681, #83310, #26023, #47314, #40213, #48263, #33599, #61567, #77165, #90400, #18455, #4257, #12295, #62025, #41140, #70073, #62990, #7525, #21271, #77640, #13713, #43511, #49220, #63457, #12791, #78117, #49680, #57736, #58211, #20810, #86122, #64408, #43054, #29318, #14655, #78575, #93235, #72409, #36410, #42565, #28388, #13255, #21751, #86581, #27930, #79517, #57280, #50143, #41632, #71481, #65325, #42092, #92287, #70551, #71007, #6613, #50627, #87056, #35493, #79041, #14193, #71958, #48736, #430, #7076, #35949, #5674, #34549, #64868, #93694, #6138, #27444, #56336, #56820, #85198, #28850, #20348, #35010, #63925, #92763, #85662, #37783, #74246, #43960, #1818, #52928, #79963, #30235, #81807, #7984, #22655, #22205, #16956, #81342, #9368, #38252, #15562, #24054, #51528, #23120, #72859, #87508, #66237, #16490, #15100, #80417, #45821, #67165, #9848, #44433, #73339, #1352, #38721, #73790, #8450, #74727, #67627, #59603, #59125, #30704, #36878, #65793, #903, #60526, #29785, #58664, #51075, #2298, #66690, #52003, #31181, #60066, #37329, #88904, #31636, #88453, #87969, #2755, #80889, #44888, #23600, #8906, #52468, #24520, #10304, #61917, #76592, #90753, #69024, #54794, #83206, #12183, #89843, #25005, #4156, #75191, #90301, #89362, #68556, #11254, #61471, #25453, #69482, #33026, #53876, #25911, #32096, #41026, #3693, #18835, #76122, #62392, #75649, #39174, #48150, #26400, #4612, #82742, #40567, #33486, #77054, #18353, #54332, #33973, #47211, #40109, #53401, #17895, #83673, #32578, #47690, #11714, #68085, #82286, #91235, #46748, #55288, #60998, #84142, #10772, #19291, #69952, #5094, #39632, #17437, #46287, #3210, #53022, #88545, #61097, #3301, #1912, #82380, #10864, #2848, #76217, #37876, #38813, #2394, #39727, #3785, #59701, #30802, #9940, #10399, #88997, #67717, #46838, #17530, #75280, #23693, #25092, #68650, #74339, #31729, #31271, #82833, #39264, #66782, #45438, #52557, #68180, #25544, #81434, #17053, #9463, #46380, #38348, #75741, #32192, #54425, #32669, #60620, #89936, #53966, #16582, #89458, #17986, #24619, #53504, #61555, #81900, #90388, #83296, #18444, #60158, #47302, #67261, #24144, #45918, #74826, #41128, #34538, #56808, #69580, #70061, #84238, #62495, #5202, #26496, #4708, #41619, #92277, #20798, #6128, #84707, #34999, #11809, #11347, #12284, #63915, #85650, #40660, #49668, #5662, #13244, #91334, #4243, #55387, #62978, #33586, #19854, #42080, #33123, #69117, #62012, #40201, #90847, #26009, #54895, #27433, #26963, #34076, #56325, #20337, #83772, #85189, #18928, #48725, #47783, #76684, #19388, #48251, #12777, #49207, #77153, #91811, #55854, #77627, #78103, #70540, #63446, #70996, #92752, #27920, #86111, #21260, #72397, #35481, #28841, #78564, #64856, #14644, #57725, #86572, #15089, #7515, #50130, #65314, #57267, #87496, #93683, #87046, #43501, #7974, #71947, #93223, #29775, #36400, #42554, #21741, #892, #79029, #64397, #71471, #14183, #50617, #43949, #51517, #79507, #421, #29308, #58202, #13702, #58654, #22195, #51064, #22645, #6603, #79951, #72846, #36868, #28376, #43044, #65783, #7067, #35938, #26333, #33423, #20165, #63283, #6432, #85013, #27749, #91166, #49046, #35307, #62326, #77459, #64233, #55226, #69888, #69418, #93063, #34840, #56645, #92580, #62817, #71303, #5027, #70380, #84080, #40966, #19688, #63751, #19230, #33908, #28219, #85495, #57107, #91650, #26804, #48557, #85947, #27270, #55690, #21099, #49967, #13085, #12602, #77941, #4549, #5507, #78858, #14008, #84541, #48088, #20642, #76992, #41448, #12121, #34378, #56157, #92116, #41923, #70834, #5966, #49512, #78404, #13543, #42391, #30523, #65617, #72689, #81176, #729, #58493, #42868, #7351, #44252, #50908, #66073, #1185, #86406, #71782, #30066, #43340, #22039, #14482, #8736, #72237, #15387, #80251, #37164, #86885, #36233, #66524, #6904, #58031, #93518, #58951, #8284, #35779, #87338, #15868, #7808, #64692, #28677, #43789, #65151, #44724, #37613, #57563, #21560, #14934, #73164, #254, #36697, #51822, #22487, #87799, #50444, #22948, #73624, #79347, #29615, #29136, #80714, #1643, #79792, #51360, #59423, #88275, #23431, #52299, #89193, #23884, #24826, #52752, #54162, #82577, #32857, #83031, #82102, #89657, #68378, #45172, #75023, #61299, #46120, #67916, #11066, #31468, #46579, #17261, #10136, #74543, #18185, #17724, #74074, #90134, #53710, #39002, #39461, #61746, #9674, #3040, #24346, #67459, #31923, #60356, #38557, #75477, #3508, #25738, #39936, #10602, #68853, #16781, #81634, #90578, #53221, #32400, #60815, #47037, #2588, #59896, #3982, #25285, #9193, #75938, #54620, #45635, #31009, #38071, #16320, #66981, #2119, #88738, #55584, #27158, #5403, #77827, #64116, #49407, #19580, #34268, #78297, #13436, #84432, #63175, #47979, #56531 ),
 ( #92467, #92005, #56046, #40391, #70726, #20537, #26215, #48449, #76883, #34729, #84900, #18649, #91043, #11544, #20049, #71195, #28113, #62708, #55110, #48929, #83976, #27633, #12977, #6322, #85388, #77350, #41815, #5858, #47516, #12484, #63645, #41334, #70269, #42283, #4908, #35190, #92953, #83492, #12010, #76422, #69309, #4437, #33317, #62213, #19124, #40860, #69778, #33793, #91538, #26695, #15629, #52074, #73404, #22718, #88517, #45410, #67690, #52997, #37848, #81871, #58729, #57001, #59190, #17022, #9913, #87574, #38786, #52531, #60131, #44498, #1882, #81406, #8514, #51593, #45891, #20989, #37393, #13896, #16555, #23665, #49856, #8970, #31244, #23193, #2818, #85838, #88036, #80479, #88970, #24117, #78755, #42750, #30303, #30775, #66302, #80957, #67236, #66754, #59674, #71666, #74309, #74796, #93414, #16101, #1416, #9435, #38322, #6800, #64589, #35674, #2366, #29846, #44953, #73853, #39234, #40167, #68151, #69542, #4212, #48211, #4673, #3754, #11316, #83738, #60593, #90357, #76648, #61526, #83266, #26461, #46807, #61977, #32636, #25514, #89905, #33547, #33087, #89428, #11773, #69084, #54392, #54856, #77114, #25063, #18410, #10833, #82804, #47270, #75710, #53935, #90813, #18895, #41090, #55350, #25972, #84202, #32163, #31700, #76186, #19349, #12244, #61064, #70018, #47750, #62455, #17955, #24584, #39695, #40626, #68620, #91298, #53472, #82351, #17499, #46352, #75253, #10368, #3271, #27884, #34964, #43461, #56774, #20762, #5161, #63411, #6565, #13209, #28341, #57231, #48683, #34036, #86073, #5629, #78066, #70502, #64819, #34504, #71430, #49634, #92714, #35901, #78529, #21223, #26925, #13667, #93643, #62939, #42044, #28802, #84665, #92239, #91773, #57687, #64363, #50093, #78987, #27395, #7031, #56285, #6091, #55812, #85148, #49173, #93189, #19817, #20301, #86530, #14142, #21697, #70959, #63876, #85616, #50574, #42519, #35444, #79469, #14603, #43006, #71910, #77587, #12738, #41580, #378, #16909, #29267, #65273, #72358, #59553, #87919, #8404, #88403, #81297, #58162, #23553, #81758, #51949, #15051, #24006, #855, #87006, #73744, #52422, #36360, #7475, #22158, #44841, #16443, #8856, #80840, #37734, #66188, #88857, #72808, #7933, #15989, #51026, #73292, #79914, #51480, #23070, #44382, #37282, #45295, #66641, #36827, #1768, #43912, #52879, #80368, #30652, #59075, #74199, #58617, #65746, #31132, #9317, #29736, #1305, #67114, #87458, #22605, #15509, #30187, #38200, #2248, #60018, #17847, #83152, #61422, #40060, #26349, #11667, #75600, #90254, #40516, #69434, #46698, #25403, #10256, #18783, #54743, #24953, #76544, #54282, #2708, #9801, #45767, #10723, #4564, #91182, #75144, #55241, #68977, #47641, #32047, #38675, #60941, #3638, #39124, #18303, #33438, #62341, #25861, #68036, #90701, #83621, #84097, #68503, #39580, #74677, #32528, #47161, #67580, #3162, #76070, #53830, #4107, #32979, #89315, #31590, #61870, #46240, #82696, #17391, #60479, #89790, #11201, #24470, #53350, #82235, #12617, #42883, #77008, #34392, #69903, #42407, #78419, #12136, #63766, #85961, #77956, #57576, #19246, #20180, #77474, #21112, #78873, #40981, #5042, #85029, #85509, #70394, #49060, #28232, #92596, #56660, #33923, #6448, #49980, #55705, #13099, #41463, #64248, #20656, #48104, #26819, #62831, #49526, #6918, #91665, #92130, #84556, #27765, #19703, #57120, #13557, #35792, #14022, #41937, #71317, #35323, #48573, #70849, #93078, #5982, #34854, #71796, #63299, #64705, #93532, #28690, #5522, #27285, #56172, #21576, #66540, #30084, #22505, #15884, #38089, #50924, #51376, #747, #43804, #80267, #7823, #79808, #22965, #73642, #2136, #81192, #66089, #16338, #86900, #51838, #8752, #31025, #45188, #1202, #74091, #22055, #86420, #87355, #9210, #66999, #72704, #50458, #80731, #88292, #36713, #79361, #29631, #44271, #58510, #58968, #23447, #52315, #1660, #15404, #37631, #30540, #14496, #73181, #8300, #43354, #37182, #87815, #72250, #44740, #59441, #7367, #36248, #65166, #271, #29152, #58049, #60372, #39018, #31484, #25753, #89211, #32414, #3523, #54177, #10151, #53239, #83507, #23900, #75039, #16798, #83047, #25299, #52771, #10616, #32872, #24843, #4451, #59912, #60831, #24362, #61760, #54634, #81650, #45653, #31941, #61313, #17279, #89675, #68867, #39474, #90151, #74561, #47051, #90593, #2604, #53726, #82121, #11084, #18199, #88754, #67475, #9691, #75953, #47532, #38572, #67933, #46136, #68393, #3056, #3997, #39951, #76436, #18665, #82592, #11557, #40405, #17739, #46593, #69323, #75492, #84913, #28126, #48463, #63658, #34281, #5416, #91552, #35206, #5873, #62227, #13449, #70739, #63189, #56546, #78769, #26709, #92019, #12498, #84445, #27172, #77363, #55597, #57015, #56060, #77842, #19594, #6336, #42299, #41350, #64134, #12990, #83990, #91057, #41828, #20062, #92968, #48943, #85402, #55125, #34742, #85851, #26231, #70283, #21004, #19137, #33809, #33330, #49870, #92481, #20550, #49420, #27647, #13910, #62722, #78310, #47992, #4923, #71209, #42764, #76896, #71683, #12025, #40873, #69791, #65056, #36138, #50816, #23324, #58398, #72145, #30424, #59315, #44150, #79700, #15293, #28580, #64602, #57471, #45072, #86313, #93428, #6814, #87699, #22390, #36598, #22851, #15764, #21465, #51717, #16221, #80154, #43247, #52195, #29037, #50340, #8186, #80606, #79246, #35688, #14388, #73056, #44624, #37068, #65977, #1088, #633, #81077, #7261, #158, #29969, #57927, #7714, #86784, #14842, #51262, #72593, #65514, #73526, #58854, #21943, #8635, #43695, #29518, #87244, #37512, #66422, #1540, #88165, #23783, #32756, #46472, #9088, #38901, #68748, #74431, #88635, #37966, #9561, #74920, #82925, #83387, #46016, #17621, #89551, #68274, #54517, #39824, #10031, #24718, #3878, #53603, #73972, #38449, #75376, #81995, #3396, #32286, #52647, #66874, #61192, #67356, #53115, #45530, #61644, #2486, #10489, #39357, #90029, #24240, #31363, #90477, #2010, #89089, #30903, #25181, #54055, #59794, #82474, #46931, #67810, #18537, #81527, #2935, #60252, #75834, #25634, #16674, #17150, #31820, #18078, #60712, #10957, #56421, #91898, #84794, #4336, #34629, #78195, #83869, #12375, #11905, #92366, #48816, #76314, #54996, #69207, #19945, #35090, #85743, #26587, #19021, #55939, #47875, #85281, #77721, #64009, #20431, #19476, #27052, #5755, #11440, #41222, #27528, #77245, #5296, #42175, #62591, #12872, #48343, #70160, #40754, #49300, #41711, #40291, #13334, #70628, #34166, #63540, #92847, #69671, #63068, #55477, #4803, #71088, #91435, #33683, #6221, #28011, #56903, #47403, #33213, #62108, #76778, #90940, #26104, #84326, #66319, #50225, #1434, #15185, #22736, #7157, #13797, #36032, #72487, #79129, #518, #51609, #80498, #982, #14276, #65873, #29863, #8530, #43591, #50707, #59208, #7603, #14736, #64949, #43136, #51158, #8071, #30318, #15646, #29401, #44515, #21354, #20890, #21832, #73420, #49762, #72041, #78657, #44044, #37409, #50, #42649, #28930, #36490, #57817, #58293, #71566, #6701, #58748, #86668, #87590, #35575, #64491, #65407, #79595, #93317, #87136, #22287, #28469, #80045, #72946, #36960, #57362, #86204, #37866, #88054, #75271, #88534, #67251, #59691, #53955, #23682, #60609, #31718, #82369, #38338, #81423, #17975, #52091, #9452, #44969, #17519 ),
 ( #80974, #52547, #82822, #10388, #75729, #16572, #45427, #2382, #10852, #45908, #74327, #46827, #39716, #89446, #31261, #2836, #16118, #73870, #8987, #32657, #66770, #1902, #23211, #39253, #9929, #24134, #68168, #3289, #30792, #32181, #3772, #67707, #60148, #68640, #88987, #53012, #24605, #61084, #81888, #17042, #74814, #53493, #89925, #38803, #46369, #25081, #85975, #21125, #12632, #61545, #49993, #63313, #41950, #34406, #28703, #92144, #35336, #6462, #57133, #13114, #56186, #86432, #25534, #77972, #19717, #78888, #28246, #54414, #13570, #35804, #27779, #7379, #90378, #63780, #27299, #64717, #57588, #84570, #48588, #34867, #64262, #20194, #92609, #71809, #42420, #93092, #77488, #14035, #93544, #5535, #56673, #85045, #42896, #6931, #41478, #70410, #49073, #21591, #50470, #70863, #5994, #85522, #71332, #20667, #79373, #14510, #43366, #72262, #49539, #78433, #88303, #65180, #1213, #81204, #66101, #87827, #31037, #51387, #66550, #37194, #8311, #758, #38103, #8763, #284, #16350, #73653, #30095, #59452, #81662, #29643, #58979, #15417, #87366, #22978, #80278, #58522, #1672, #23460, #45667, #59927, #15895, #88766, #36725, #36260, #51851, #23912, #16810, #65644, #74575, #30554, #67013, #22516, #29164, #44285, #80744, #73192, #44752, #2148, #52784, #45200, #37642, #74103, #9222, #58060, #52327, #86912, #22067, #50935, #79819, #14960, #43815, #72715, #7838, #38584, #17292, #31496, #75971, #91077, #48008, #82605, #46148, #18215, #75052, #47546, #11100, #26248, #76450, #75507, #83061, #61774, #67487, #68410, #54650, #39487, #61327, #4468, #24855, #39965, #10629, #3539, #67945, #11571, #68881, #2618, #83524, #47065, #32428, #32887, #55141, #3068, #90165, #17752, #60846, #25313, #53739, #31953, #4011, #90607, #19152, #33345, #25768, #62242, #10163, #9703, #54192, #84004, #60384, #39032, #89223, #18682, #40419, #89689, #24374, #46605, #69337, #53253, #82135, #13926, #42784, #57031, #70301, #28142, #85869, #64617, #5890, #13009, #21480, #34760, #92498, #76912, #41367, #78326, #84930, #6352, #35225, #26726, #12042, #64151, #77379, #56077, #48480, #71701, #12517, #49438, #20566, #71225, #27190, #5432, #6829, #40889, #92035, #33829, #92984, #42316, #69807, #27667, #49888, #41845, #4943, #62738, #77859, #34298, #78785, #35703, #91569, #55612, #48963, #13466, #63205, #70757, #21020, #56565, #93443, #84461, #28597, #57487, #19611, #63675, #86329, #85418, #20082, #14858, #23342, #59331, #29533, #81092, #1103, #7276, #14403, #29984, #44167, #16236, #65992, #8649, #72160, #58868, #45086, #43262, #58413, #73987, #36153, #50832, #50358, #9104, #15780, #37526, #73540, #43711, #52210, #79716, #51277, #65075, #21959, #650, #44638, #174, #72610, #37981, #66436, #66889, #7732, #36613, #87259, #2028, #8204, #65533, #30919, #59809, #87715, #22405, #22866, #29054, #57946, #86801, #88650, #80170, #15308, #79263, #1556, #51731, #73073, #30439, #88182, #37083, #80624, #33226, #3410, #60267, #69220, #46032, #38467, #25195, #10970, #81542, #52662, #67371, #90043, #39838, #54069, #32303, #82939, #17637, #40305, #24256, #53130, #61208, #9578, #24736, #23798, #2951, #39373, #89566, #53619, #3892, #18091, #82010, #46945, #89104, #4349, #31837, #75847, #10504, #90489, #10047, #2500, #76328, #68762, #16690, #82489, #18550, #17167, #31378, #45545, #74937, #46488, #32769, #62122, #75391, #61657, #68289, #25648, #74446, #83400, #54531, #47418, #11453, #38917, #67826, #60727, #84339, #92860, #26600, #91911, #19034, #62607, #41235, #56431, #55011, #91450, #56913, #78206, #78668, #55490, #19490, #70175, #13809, #48828, #48356, #20901, #49773, #34641, #5310, #5767, #47888, #83884, #76792, #35588, #11918, #40767, #90953, #13345, #12886, #27065, #42186, #6232, #69685, #71099, #6714, #70639, #33696, #42661, #77259, #4815, #92380, #35102, #12389, #26117, #34179, #63551, #64020, #27539, #85294, #20444, #84807, #71578, #63081, #55952, #49312, #19957, #77735, #41723, #28024, #85754, #36501, #65417, #44527, #72955, #64960, #36971, #7168, #80986, #72497, #87601, #51168, #37420, #50720, #14288, #23221, #65885, #93328, #29413, #59219, #61, #79139, #28479, #28942, #528, #73431, #73880, #58304, #8083, #80055, #58759, #44979, #30329, #87147, #15195, #88064, #52101, #22297, #44055, #57828, #66331, #8541, #43601, #1444, #994, #21366, #57372, #29875, #22747, #16128, #51622, #80509, #86214, #15657, #8998, #50236, #7614, #64502, #43149, #86678, #72052, #36043, #21843, #79605, #14746, #7581, #16545, #87113, #79570, #66294, #52065, #28905, #26, #14713, #37384, #80947, #1406, #44491, #30293, #58721, #81397, #65381, #493, #73395, #50684, #65851, #64923, #44019, #80470, #36937, #959, #44944, #8505, #29377, #59181, #36466, #45401, #72916, #88025, #51584, #37839, #51137, #43566, #23655, #23182, #57793, #29838, #59665, #58271, #72462, #86643, #22263, #87565, #73844, #74300, #22710, #16092, #15619, #8960, #9424, #30763, #66745, #1871, #88508, #52521, #21810, #80020, #15160, #8043, #47262, #17490, #69077, #82795, #88960, #2357, #17947, #32153, #4205, #53927, #90349, #60121, #46798, #33080, #31235, #46342, #61969, #24107, #38777, #38311, #90806, #3746, #25505, #61518, #31689, #40160, #67681, #39224, #52988, #9903, #82342, #32628, #81862, #2807, #25965, #54383, #54846, #60584, #89419, #75244, #83728, #89897, #24573, #18888, #47743, #75700, #10359, #10825, #17011, #45880, #74786, #76641, #53461, #68142, #67226, #83259, #39685, #3263, #18403, #76176, #61054, #25055, #68609, #11308, #26454, #69534, #12237, #12729, #20754, #21213, #77578, #49166, #27388, #6083, #86063, #71422, #41572, #56278, #6554, #35433, #70494, #85137, #70008, #78521, #49625, #84657, #42510, #20292, #62445, #4667, #78059, #5622, #64355, #13201, #63869, #33540, #42037, #93181, #91288, #19809, #28333, #55343, #41084, #11766, #57223, #70951, #92703, #34957, #5151, #13658, #34028, #34497, #84194, #77106, #55805, #27873, #19342, #62932, #50083, #56766, #40618, #91766, #26918, #48677, #48204, #63403, #92232, #85607, #8847, #22595, #58151, #87449, #7021, #42995, #35892, #23543, #64810, #71901, #78978, #66179, #846, #15042, #1296, #87910, #93634, #30178, #88392, #58608, #21686, #30643, #7466, #28791, #80359, #59062, #57678, #14130, #86521, #51470, #23061, #15500, #44371, #73282, #72799, #1756, #79460, #14594, #8395, #50563, #79904, #43451, #86997, #29727, #51017, #43902, #51939, #37273, #72348, #80829, #36349, #59542, #22149, #15980, #65735, #44832, #65263, #369, #37725, #73735, #29255, #7923, #36814, #66631, #24942, #9791, #82225, #61412, #3154, #89779, #9308, #39571, #83143, #88848, #17379, #16899, #3628, #53819, #81288, #60008, #74189, #82687, #40050, #90692, #31581, #23997, #60932, #52870, #90244, #17837, #68967, #25393, #24461, #32037, #10714, #16434, #46231, #32516, #75135, #10245, #47152, #67570, #46689, #53340, #39114, #45757, #54273, #75591, #45286, #18294, #68493, #68027, #76061, #4097, #74667, #11190, #60470, #38666, #32968, #2699, #89305, #61861, #52413, #38190, #67104, #2238, #31122, #81749, #25852, #26809, #78409, #71308, #55231, #6438, #20171, #27755, #12126, #18773, #40972, #77465, #84086, #5513, #56651, #85500, #5972, #19236, #70839, #34845 ),
 ( #20647, #70385, #76535, #83612, #34383, #19693, #49517, #41453, #77946, #47631, #63288, #13548, #11657, #33913, #42397, #40504, #26338, #49051, #35313, #69894, #69423, #5033, #12608, #48093, #92121, #64238, #54734, #63756, #76997, #92586, #4554, #33428, #48562, #55695, #62332, #27275, #56162, #91172, #62822, #85019, #91656, #13090, #41928, #84546, #93069, #80257, #93522, #72241, #64696, #58957, #28681, #65624, #36703, #87344, #43344, #86410, #22954, #57111, #14486, #49971, #22493, #58499, #85951, #43794, #66079, #58038, #37619, #28223, #259, #57567, #1191, #87805, #21103, #78863, #65156, #736, #50449, #29142, #8290, #72694, #29621, #14013, #15393, #30072, #35783, #86890, #21566, #44260, #51366, #42873, #6908, #71786, #73171, #80721, #79351, #7356, #36238, #7813, #22044, #37171, #51828, #15874, #44730, #50913, #73631, #8742, #79797, #14939, #17730, #2594, #24352, #61304, #81640, #3046, #67465, #38563, #31015, #68383, #39008, #1649, #46585, #10142, #31474, #89664, #18190, #59902, #60362, #45641, #23890, #89200, #16787, #88744, #31930, #53716, #75943, #90140, #46126, #25290, #66988, #66530, #53227, #54168, #47042, #2126, #11073, #52759, #82109, #75483, #17268, #67922, #23437, #82583, #3514, #9199, #75029, #74550, #10608, #60821, #30529, #74080, #88282, #24833, #83037, #59431, #9681, #38077, #39466, #32406, #52305, #81182, #16328, #45178, #13320, #20876, #93305, #68858, #6209, #86190, #71077, #92835, #36018, #56408, #71552, #42160, #35077, #5742, #43124, #13785, #3987, #21342, #78645, #63996, #64477, #86655, #34617, #27998, #20418, #92354, #56890, #85269, #63527, #6689, #28455, #50695, #64936, #49748, #37, #41697, #39942, #85730, #28917, #21820, #70615, #79582, #35564, #72028, #27514, #32862, #49286, #42636, #78182, #57350, #7144, #57805, #50212, #79116, #14264, #61751, #90583, #25744, #54625, #83497, #18655, #47522, #76427, #12859, #16105, #22722, #37855, #66759, #58281, #14724, #1888, #15172, #87578, #80031, #74316, #44030, #80961, #52078, #8975, #58735, #8057, #38327, #72475, #29851, #65393, #30780, #73857, #7591, #59194, #81411, #73408, #53002, #43577, #15633, #72931, #16561, #9440, #36477, #506, #80484, #44957, #29389, #51597, #45416, #87123, #36949, #22275, #67241, #59679, #88522, #23670, #65862, #2371, #970, #44502, #51147, #8518, #37397, #52536, #66307, #1422, #31249, #60136, #88975, #30306, #88041, #23197, #24123, #39701, #53479, #11781, #40631, #25520, #61069, #90363, #9918, #45896, #38791, #26467, #67695, #74801, #81876, #69092, #3759, #17960, #4218, #90819, #2823, #33093, #91304, #61532, #24590, #33553, #10373, #31705, #83272, #61984, #60598, #17030, #89433, #54399, #25978, #18416, #47276, #76192, #75715, #4679, #82356, #17504, #11322, #46357, #82809, #75258, #89912, #32644, #53940, #46813, #54863, #40173, #39240, #83744, #68156, #62462, #25068, #18901, #68625, #47756, #3276, #32168, #69549, #76654, #10838, #20307, #50098, #55818, #70024, #19355, #84674, #56291, #64368, #64824, #27403, #92719, #70965, #49639, #35906, #21229, #85154, #6097, #78992, #14147, #49178, #34969, #19823, #28346, #93194, #34510, #86078, #63883, #12250, #48219, #27889, #78072, #43011, #56779, #13673, #77121, #85621, #71915, #63417, #12744, #13215, #70508, #48689, #20767, #42523, #93648, #7036, #78534, #55356, #77594, #84208, #42051, #41096, #5167, #41586, #34042, #71435, #57236, #5635, #62945, #92246, #6571, #35449, #91779, #26930, #59559, #8862, #22164, #73750, #37740, #16449, #51486, #58623, #67120, #80374, #44389, #28808, #87012, #30193, #36833, #51955, #80847, #72364, #57692, #15995, #29272, #7940, #384, #88409, #58168, #1311, #66195, #23076, #72814, #51032, #52428, #86535, #43919, #79475, #44847, #87925, #21703, #73298, #1774, #87464, #50580, #14609, #29742, #79920, #30658, #23560, #43467, #7481, #861, #59083, #15057, #22611, #66648, #8410, #81303, #36366, #45301, #74206, #65279, #15515, #65752, #9323, #38206, #37288, #9806, #24011, #68509, #83627, #40522, #75149, #38680, #10730, #67585, #40065, #3644, #18789, #68983, #68042, #75607, #54288, #31138, #60947, #47167, #32053, #53836, #90707, #17396, #32535, #3169, #89797, #60484, #4113, #61428, #60025, #76076, #39586, #24960, #25409, #47648, #89321, #82702, #90260, #17853, #83159, #76550, #24476, #46704, #10261, #53355, #18311, #46245, #82240, #11207, #32985, #11673, #25868, #61876, #54750, #2715, #2255, #88862, #52884, #81764, #31595, #16914, #45772, #74682, #39131, #62347, #55711, #27291, #5048, #49066, #6453, #35328, #49531, #62838, #20660, #78424, #57125, #92136, #5528, #14027, #56178, #85036, #69440, #33930, #70855, #77480, #92601, #27771, #19252, #4570, #56665, #69909, #48580, #40988, #64254, #91671, #41943, #13106, #63772, #19709, #26824, #93083, #33444, #84562, #26355, #85514, #34859, #91188, #20186, #42412, #34398, #55246, #84103, #70401, #12623, #71323, #28238, #48110, #77014, #41469, #5987, #63305, #77963, #13562, #85967, #21117, #12142, #49985, #78879, #79366, #7830, #7372, #87821, #44277, #71801, #50463, #64710, #15410, #30547, #81198, #22060, #14502, #51381, #43359, #80737, #73186, #59446, #15889, #14954, #22510, #1207, #6923, #36719, #22971, #72709, #752, #37636, #58054, #8305, #43809, #65639, #36253, #44745, #37187, #35797, #51843, #30089, #88297, #65172, #72255, #86905, #23453, #29636, #277, #66544, #1665, #80272, #50929, #66095, #93537, #28696, #57581, #42888, #86426, #21581, #29157, #58973, #58515, #87360, #73647, #8757, #79813, #52320, #25759, #89682, #52777, #61766, #38578, #31031, #17745, #3530, #74097, #45194, #59919, #82598, #32420, #46599, #24849, #75499, #10157, #32878, #16804, #45660, #53732, #2142, #17285, #16344, #89217, #31947, #82128, #46142, #90157, #10622, #74568, #39480, #81656, #90599, #24368, #68401, #3062, #83053, #2611, #88760, #68873, #61319, #9216, #75045, #11091, #9697, #23906, #38096, #67481, #39025, #25305, #54641, #67939, #54183, #60839, #18206, #67006, #75961, #47057, #39957, #4003, #31490, #60378, #53246, #55132, #20072, #84921, #40880, #77850, #19602, #76442, #18672, #48470, #91559, #12999, #84452, #63196, #11563, #77370, #41836, #47538, #69798, #70747, #40411, #91067, #83515, #63666, #56068, #48952, #5881, #4932, #92489, #12033, #12507, #62234, #76903, #26716, #34751, #4460, #33818, #27657, #69329, #62729, #55603, #92026, #83996, #41358, #33337, #70291, #27181, #5423, #34288, #26239, #19144, #47999, #46892, #17107, #90897, #82432, #3837, #61152, #47357, #60672, #24197, #33173, #75793, #9517, #39316, #69167, #74879, #89048, #38405, #9989, #75334, #83346, #83828, #46431, #18040, #89987, #68707, #54950, #40251, #10450, #25141, #4294, #62063, #68233, #54017, #38862, #76273, #18493, #53560, #11399, #82884, #31322, #67314, #10915, #3354, #26061, #39783, #32719, #2444, #61604, #18982, #60209, #17582, #74389, #53074, #67768, #81950, #45973, #90437, #25594, #54477, #2895, #31778, #89509, #32244, #24674, #19438, #91860, #13295, #11863, #48303, #13761, #35050, #35537, #12333, #77203, #27014, #64451, #5716, #41178, #71525, #6659, #85243, #55902, #56377, #69632, #40713, #4760, #86163, #33641, #62550, #47834, #63966, #63499, #77681, #92807, #56863, #91393, #27973, #57322, #27485 ),
 ( #84755, #71050, #6183, #26548, #76736, #85705, #70118, #19903, #5256, #42609, #34125, #20391, #49262, #42133, #48775, #63029, #93277, #55436, #12833, #84288, #20850, #49721, #41671, #92329, #78617, #70589, #34591, #78157, #28429, #79556, #23167, #80934, #43096, #79085, #87099, #87549, #72448, #51119, #30277, #65838, #58706, #72001, #8492, #52050, #57779, #80005, #14697, #66280, #22696, #50187, #28890, #7120, #51571, #8947, #59651, #476, #86625, #29824, #21795, #59167, #80457, #37826, #88013, #22249, #946, #73382, #14237, #15144, #1393, #44005, #72903, #16079, #36452, #15604, #8027, #36923, #43552, #44932, #44476, #35989, #73833, #37370, #66732, #1859, #30749, #7567, #21315, #29364, #65367, #64909, #58256, #11, #50670, #75689, #4195, #83248, #68128, #18394, #88948, #88496, #89407, #47251, #40150, #24095, #69066, #82784, #90340, #74772, #81385, #9890, #46330, #52974, #3252, #25495, #54373, #68598, #81849, #39676, #16999, #61040, #32142, #17936, #38765, #45866, #76164, #52509, #67669, #45386, #46787, #53916, #16533, #39213, #61508, #53447, #33070, #23643, #24561, #2795, #11297, #74287, #9411, #38297, #60571, #89884, #31677, #82329, #3734, #25044, #10814, #67211, #32618, #2344, #31223, #17479, #75233, #60108, #10347, #90796, #69524, #83716, #34485, #49612, #6542, #41073, #4655, #70482, #33529, #6070, #63391, #78507, #34943, #34017, #41559, #20277, #25955, #26907, #13189, #91755, #19798, #56751, #77096, #92221, #62920, #55795, #26442, #63857, #27376, #54836, #42024, #5610, #84647, #85126, #13645, #55333, #48667, #69998, #19332, #77568, #12226, #84184, #56266, #49152, #71410, #85594, #78048, #20741, #62435, #61960, #12717, #42496, #18877, #91276, #47733, #70939, #92690, #48194, #76632, #5138, #27860, #11756, #40608, #67446, #2574, #16767, #28778, #81618, #45621, #24330, #59406, #66508, #75010, #88259, #52283, #35419, #93620, #38056, #44709, #59882, #88722, #78965, #64340, #23870, #35879, #15851, #7007, #31452, #52736, #66965, #16307, #2103, #30510, #53207, #64796, #57662, #45159, #21198, #37598, #93167, #73610, #81163, #8720, #1628, #74523, #74058, #86509, #9178, #71885, #82085, #23418, #9657, #30995, #38543, #21672, #14116, #89178, #60341, #28319, #17243, #46105, #51806, #50069, #57208, #80698, #86049, #42979, #19567, #75924, #47500, #25723, #4424, #84419, #69764, #39920, #54607, #4895, #33779, #11050, #83478, #68363, #76870, #19111, #83017, #40845, #18634, #60802, #67901, #76409, #3969, #62692, #11531, #62200, #31910, #40378, #91525, #3024, #18169, #26681, #89640, #10584, #10122, #55571, #69295, #91030, #33302, #3491, #11996, #39447, #68841, #24810, #75463, #54148, #26199, #53696, #32384, #48433, #55093, #38988, #61285, #90119, #47022, #82563, #61733, #25271, #17711, #46564, #83962, #32843, #47966, #90565, #41318, #5390, #21916, #34255, #70255, #77337, #64577, #92940, #13423, #93402, #86286, #63161, #28554, #86754, #56988, #20036, #29013, #5845, #91992, #78740, #57445, #27145, #12471, #56030, #49844, #35662, #84885, #42268, #21439, #71181, #35178, #72121, #92456, #13884, #78285, #49393, #41803, #79218, #42737, #48913, #50313, #20977, #6310, #6785, #57898, #70714, #64100, #56516, #34717, #28101, #27619, #63631, #71652, #14360, #77815, #7237, #85826, #36112, #12964, #85375, #43220, #65030, #20525, #130, #2462, #45046, #52621, #37039, #43671, #65953, #8611, #80125, #30399, #81503, #16650, #30875, #44124, #1984, #59769, #38421, #73499, #80581, #89064, #37487, #66397, #50790, #15264, #52168, #58828, #73947, #9062, #605, #14816, #37940, #51237, #29943, #22363, #45504, #73028, #23295, #88137, #66849, #1064, #8156, #74406, #72566, #87673, #7688, #88610, #16194, #36573, #1513, #9536, #15734, #65488, #29488, #51692, #22823, #67330, #31338, #58373, #87215, #44595, #81051, #59291, #60225, #33190, #68722, #61621, #74895, #11415, #54968, #60688, #82899, #82450, #69183, #25610, #53089, #31794, #45990, #90453, #11880, #62567, #3373, #89528, #54493, #24692, #62080, #83361, #40731, #90913, #90003, #3852, #47850, #81968, #39331, #10006, #47375, #18511, #17124, #76289, #26079, #18055, #24214, #38877, #25158, #17598, #83844, #18997, #67784, #2910, #54032, #40266, #75350, #46907, #76752, #4312, #69648, #53575, #4776, #33658, #46448, #75808, #10465, #68249, #32261, #61167, #10932, #39800, #63984, #79103, #36005, #70603, #5271, #6197, #34140, #35552, #92824, #14252, #64465, #63515, #71065, #49735, #26563, #56396, #42623, #27498, #49276, #86178, #12847, #27987, #92343, #85258, #55917, #93292, #56878, #55452, #71542, #35064, #20406, #20864, #43110, #84769, #78171, #5730, #48790, #13309, #41685, #19918, #85719, #78632, #7134, #21329, #13774, #50199, #91874, #91408, #42147, #72017, #84303, #27028, #19453, #6675, #28443, #77698, #48319, #34605, #57336, #77220, #12348, #41197, #70135, #63043, #67379, #26495, #55386, #62977, #4242, #11346, #19853, #33122, #90846, #9113, #38475, #76683, #82019, #4707, #33585, #23807, #37989, #62494, #74454, #53139, #45554, #41127, #9587, #47782, #18927, #69579, #24264, #2509, #54894, #91333, #66897, #40200, #84237, #69116, #62011, #70060, #89113, #11808, #76216, #47301, #31386, #77152, #40659, #2037, #19387, #48250, #26008, #12283, #26962, #60276, #83771, #18443, #5201, #34075, #91810, #55853, #84706, #30927, #59817, #88658, #52670, #81551, #16699, #48724, #49667, #7514, #420, #78102, #29307, #43043, #50616, #34998, #41618, #63914, #6602, #13243, #28375, #79506, #14643, #28840, #42079, #93682, #57724, #36399, #71470, #78563, #87045, #35480, #64396, #77626, #70995, #50129, #56807, #71946, #7066, #92276, #12776, #35937, #49206, #27919, #20336, #43500, #6127, #21259, #86110, #64855, #92751, #85649, #72396, #70539, #20797, #5661, #86571, #14182, #34537, #93222, #21740, #13701, #63445, #27432, #42553, #57266, #65313, #58201, #56324, #85188, #79028, #88442, #73329, #51992, #31170, #66679, #59592, #72845, #9356, #52918, #58653, #80880, #80404, #67154, #23591, #51063, #29774, #43948, #52458, #9838, #60517, #1341, #87495, #30692, #22644, #60056, #81332, #38711, #88894, #87956, #1806, #81797, #16945, #2287, #15551, #24043, #45809, #67618, #44878, #16027, #22194, #73780, #37773, #79950, #44423, #16479, #30224, #45335, #74236, #65782, #15088, #38240, #51516, #59115, #8440, #74718, #37319, #2746, #31626, #7973, #66227, #23109, #36867, #891, #8895, #46277, #18827, #54784, #53391, #40100, #62380, #54321, #33966, #89353, #90292, #53867, #91225, #55280, #17428, #82276, #61461, #61909, #46737, #25444, #4604, #69016, #33018, #75181, #76583, #26392, #32085, #83196, #82733, #40558, #90744, #24509, #3201, #10294, #25902, #77045, #39164, #68545, #60986, #4147, #89834, #33477, #83663, #12176, #84134, #18344, #47682, #11706, #68076, #47199, #69472, #76113, #11246, #19284, #10763, #48143, #41019, #69942, #17885, #5085, #24995, #75640, #39621, #3684, #32569, #86000, #14532, #27326, #92634, #41975, #20223, #56699, #77999, #56212, #93115, #50019, #72282, #57611, #42446, #86454, #63338, #62870, #63805, #21612, #43387, #92169, #7402, #57159, #64742, #49101, #55743, #13139, #20693, #85071, #13594, #28726, #50495, #27806, #71356, #70889, #35828, #71837, #6019, #93569, #6487, #19745 ),
 ( #79396, #5561, #85545, #34894, #14059, #64287, #91703, #70435, #84595, #35366, #26855, #48613, #49563, #34432, #28270, #78458, #6955, #21149, #77513, #12662, #78912, #42923, #41507, #65203, #1236, #81224, #66122, #87850, #31058, #51409, #66571, #37215, #8334, #782, #38122, #8785, #306, #16370, #73674, #30118, #59472, #81683, #29665, #59001, #15441, #87390, #22999, #80301, #58545, #1693, #23481, #45689, #59945, #15919, #88785, #36746, #36283, #51874, #23933, #16832, #65668, #74597, #30575, #67033, #22537, #29186, #44307, #80767, #73218, #44774, #2169, #52805, #45221, #37663, #74123, #9244, #58083, #88327, #52348, #86936, #22088, #50958, #79841, #14981, #43837, #72739, #7859, #61797, #53274, #9726, #90629, #10183, #40442, #83546, #3089, #54673, #18704, #91101, #32449, #39509, #48031, #61352, #25334, #38605, #67964, #11122, #17773, #32909, #25791, #82158, #67509, #47568, #39052, #82625, #75071, #69359, #31974, #75993, #47089, #4037, #53759, #60867, #33366, #2639, #24877, #60406, #76474, #68905, #31518, #54213, #11594, #68430, #89244, #24397, #10651, #89710, #4489, #62267, #17314, #46168, #75528, #39988, #46628, #3560, #26270, #83082, #55164, #90186, #84028, #19173, #18237, #41868, #41390, #28167, #78349, #12064, #84485, #4967, #49461, #64641, #21507, #56101, #19634, #85441, #48503, #21045, #13491, #93469, #49913, #48987, #56588, #35251, #40911, #70781, #57057, #13033, #34784, #71726, #92060, #42338, #77886, #5914, #70323, #78808, #71250, #69831, #85893, #20591, #63699, #6379, #28622, #5454, #92525, #84956, #34322, #27691, #27214, #63228, #64176, #93008, #86356, #6853, #13954, #35728, #77403, #76936, #42811, #57511, #33851, #12540, #62760, #91594, #26749, #20106, #55635, #36641, #8231, #79740, #30012, #81120, #22894, #79288, #30466, #87742, #80197, #73568, #2058, #14882, #15336, #29559, #7756, #44197, #65562, #43736, #80654, #37555, #59836, #45113, #58896, #74015, #50858, #50385, #51304, #9132, #30948, #72636, #88678, #44667, #52238, #675, #43287, #58440, #37109, #87286, #51764, #16263, #38009, #59362, #22432, #1584, #88214, #66920, #73103, #66018, #14430, #1130, #15809, #72184, #8677, #66467, #23370, #7300, #36180, #199, #65099, #29082, #57973, #86826, #21984, #83429, #53159, #90073, #61238, #18123, #67855, #17198, #47450, #81570, #38945, #74478, #46976, #82970, #16718, #68318, #90517, #82518, #62153, #23826, #24766, #82041, #25681, #18584, #45573, #9609, #89595, #25225, #74965, #53648, #32797, #3442, #54098, #38496, #11002, #54560, #60296, #17666, #46059, #68791, #75877, #52689, #31407, #67401, #39871, #11484, #2529, #2980, #89133, #32337, #24284, #61686, #3921, #40334, #76358, #46519, #69250, #4378, #10077, #75420, #33256, #10537, #39403, #31865, #60754, #27567, #91940, #63112, #55520, #92892, #47919, #20474, #56464, #55044, #41753, #64049, #55981, #35613, #90982, #27094, #84369, #28051, #56941, #19064, #83912, #84835, #63582, #48385, #19984, #6259, #70665, #34668, #76822, #78235, #85778, #33729, #48861, #19518, #42215, #92407, #26150, #4845, #11948, #85325, #78694, #40797, #70207, #62641, #5794, #91479, #35127, #49341, #13835, #20928, #77766, #13374, #71129, #69714, #12914, #49797, #42686, #71605, #6740, #12418, #26630, #77288, #41269, #5340, #34207, #36997, #93353, #44552, #8110, #556, #87628, #16151, #28967, #29439, #43624, #21871, #58329, #79630, #57852, #1022, #51647, #73905, #59244, #44078, #88090, #64984, #64528, #65441, #23248, #45003, #87, #9021, #58784, #66354, #50746, #57396, #14771, #22321, #86706, #72980, #1469, #30355, #73455, #72521, #15687, #8566, #52127, #87172, #51192, #28504, #80079, #15222, #86238, #7641, #65908, #36525, #22778, #80533, #14314, #21390, #37445, #29900, #81008, #36067, #50259, #79167, #43174, #72076, #7192, #81924, #31297, #61579, #1935, #53049, #53991, #47326, #17554, #74364, #83321, #60183, #52580, #39289, #25117, #30830, #66805, #81460, #10425, #82860, #68208, #46406, #3327, #31753, #54448, #38374, #67288, #75306, #23717, #38836, #37900, #17076, #53531, #9964, #67743, #18012, #32217, #2417, #61124, #9487, #18467, #45944, #89963, #24643, #10889, #24168, #16609, #90411, #46865, #59727, #2869, #32693, #89021, #45464, #88569, #74852, #60645, #75769, #76242, #89483, #39752, #82407, #68678, #3813, #25568, #41150, #55875, #71017, #35021, #12306, #84727, #69602, #78127, #20359, #84261, #42102, #19876, #62036, #69140, #48746, #5226, #6149, #26986, #63468, #33146, #77650, #63935, #4268, #19411, #92773, #90870, #11833, #11374, #27941, #70561, #92297, #34559, #4732, #13265, #40684, #70083, #26034, #76707, #55408, #5685, #54917, #33610, #56832, #27454, #85672, #62518, #91359, #48274, #20820, #63001, #26520, #49690, #40224, #12801, #77176, #41643, #83797, #18952, #47806, #34099, #91831, #56346, #85208, #49231, #1702, #15929, #67045, #88794, #71492, #37673, #50154, #9738, #38614, #23491, #59012, #88339, #6623, #42577, #35503, #24405, #64419, #93245, #78585, #2182, #30585, #44783, #31068, #23942, #28398, #59956, #89254, #59486, #21281, #31526, #8343, #57290, #81234, #52814, #86132, #13724, #79052, #52358, #81694, #16381, #45231, #74136, #73684, #2648, #14203, #44319, #9254, #73231, #80779, #37226, #87859, #38131, #51886, #8794, #16842, #45698, #66131, #74609, #1246, #60414, #23008, #67518, #66582, #30128, #39517, #3099, #12076, #25804, #82168, #18246, #48044, #53767, #67972, #17325, #82633, #54223, #62279, #62774, #25342, #90642, #68917, #47580, #33863, #19184, #83091, #4049, #76949, #40924, #47098, #32919, #17783, #26283, #91114, #32460, #84039, #61809, #10191, #46176, #54684, #76005, #69845, #83558, #11608, #75081, #18717, #4978, #39060, #61360, #91606, #31982, #46636, #53284, #60875, #76485, #40453, #69371, #75537, #55179, #10661, #11135, #89722, #24886, #3570, #4501, #68438, #90194, #39999, #33380, #14446, #84967, #56115, #70792, #43302, #35742, #36195, #92537, #64189, #42351, #21059, #7317, #86371, #56601, #71264, #21522, #50400, #27703, #6392, #20118, #93484, #64656, #5927, #57526, #35263, #77415, #84500, #93022, #20603, #79305, #28180, #78823, #48514, #57069, #72199, #19646, #34797, #65114, #12554, #27227, #26762, #55647, #85907, #13968, #49926, #49002, #28637, #77900, #85456, #41403, #92073, #63712, #42826, #70338, #13044, #5465, #71741, #34336, #41881, #49473, #78363, #63242, #13503, #6868, #23844, #52710, #37575, #73119, #8695, #22002, #57990, #50873, #38516, #79755, #86843, #217, #81138, #15827, #30029, #16282, #9151, #14896, #45133, #9629, #73586, #36657, #45595, #22447, #43752, #1602, #74034, #72651, #29097, #7773, #66486, #38029, #30485, #59381, #88232, #87758, #16739, #692, #29576, #23388, #65578, #1148, #58457, #8246, #44684, #66035, #58912, #66938, #52257, #87301, #2077, #51320, #74497, #37127, #30967, #80671, #59855, #80213, #15352, #81591, #88696, #44212, #22912, #51782, #67876, #82060, #31428, #2999, #68340, #62173, #31885, #67420, #3463, #26173, #19085, #60775, #47939, #61706, #69270, #53668, #60317, #82537, #25245, #89615, #46996, #4399, #33277, #47471, #24786, #18606, #76378, #55064, #90093, #32358, #11969, #54120, #82992, #2549, #17687, #68813, #75440, #90538, #25698, #17217, #89155, #54580, #46538 ),
 ( #10558, #24304, #91004, #32816, #83451, #11504, #39423, #83933, #61258, #18142, #53181, #38964, #75898, #40353, #46078, #11022, #76842, #74985, #10096, #39892, #3943, #84856, #57418, #92427, #12441, #64548, #93373, #78255, #20007, #49361, #62662, #4867, #91496, #79189, #26651, #33750, #40817, #28071, #56486, #70685, #56959, #49815, #55541, #85796, #50282, #20494, #77308, #86257, #63133, #84390, #42236, #20947, #19539, #69735, #48405, #13393, #78712, #71149, #6278, #35148, #34689, #21408, #41291, #70226, #64070, #5361, #34227, #91962, #92910, #28523, #27117, #48885, #56001, #13854, #77787, #42708, #71625, #12935, #6758, #41775, #35631, #5815, #63603, #27590, #85345, #87188, #15238, #59260, #7658, #58800, #58347, #22337, #14788, #66369, #1038, #43193, #44567, #65926, #51208, #22794, #52143, #79646, #80098, #65459, #72539, #44094, #36543, #43642, #87645, #80550, #16167, #88108, #8128, #30370, #50762, #14333, #72999, #81023, #45019, #575, #72093, #15706, #23265, #29459, #65003, #37012, #29916, #51662, #73470, #7210, #36084, #105, #8582, #28984, #57871, #86726, #37460, #1487, #21890, #56795, #20784, #5186, #63434, #6588, #13232, #28362, #57254, #48708, #34060, #86097, #5651, #78089, #70525, #64841, #34526, #71452, #42540, #93210, #49194, #92262, #28826, #62962, #20324, #55836, #21246, #64385, #91796, #49656, #71932, #63900, #43485, #26947, #6114, #27419, #7054, #93667, #84691, #19839, #70982, #35466, #56308, #34985, #14165, #78551, #50115, #77611, #79011, #35923, #41603, #92735, #85173, #43029, #57709, #86553, #21723, #12762, #42067, #27907, #50599, #79492, #14627, #13688, #85637, #66209, #88876, #72830, #7956, #80862, #58186, #73313, #72381, #51500, #87939, #44405, #8424, #52441, #16009, #36850, #44861, #15072, #24025, #80388, #1789, #59098, #45315, #87478, #22179, #31153, #73764, #7498, #37303, #67136, #65767, #51047, #36383, #877, #1325, #81316, #81778, #23091, #8876, #51972, #66662, #52900, #38222, #37755, #30673, #2270, #60039, #59575, #88425, #29756, #74219, #16462, #15531, #9338, #23574, #29290, #65296, #16928, #401, #79935, #43933, #22627, #67601, #25425, #76565, #9821, #53850, #11688, #31609, #46259, #45788, #40539, #11226, #33000, #68998, #39146, #47664, #75163, #46719, #2729, #17411, #89814, #40081, #38694, #10276, #69454, #61891, #33459, #68057, #3183, #24976, #62362, #3662, #32067, #4585, #91204, #83177, #82716, #54303, #60499, #89335, #24490, #84116, #53371, #82256, #74699, #90724, #61444, #75622, #25884, #54765, #60963, #83642, #55261, #18326, #17867, #26372, #10745, #39603, #68526, #32551, #90274, #47182, #76093, #4129, #18806, #28253, #28710, #85053, #56681, #34875, #13577, #93552, #78895, #49081, #63787, #14042, #42904, #20203, #92617, #77495, #85982, #57141, #92151, #50001, #27787, #69924, #77028, #85528, #13121, #71818, #20675, #71339, #41001, #49546, #6938, #12157, #27307, #35811, #5065, #19726, #19266, #64725, #78441, #6469, #42428, #12641, #21132, #48595, #77980, #33947, #84577, #63320, #35346, #62852, #41487, #57595, #64270, #48124, #70417, #5543, #56194, #91686, #70870, #34413, #26837, #55725, #93098, #41957, #6001, #14518, #50478, #43373, #31044, #72268, #79381, #86439, #73660, #8319, #22523, #8771, #1678, #7387, #37649, #2154, #66109, #29172, #38109, #14967, #36268, #87834, #66557, #65188, #21598, #292, #58986, #30560, #22985, #1222, #51859, #80285, #9229, #86921, #22074, #30104, #58067, #87376, #50944, #65652, #37201, #58531, #51395, #59458, #80751, #79827, #15903, #43823, #67019, #766, #44760, #73199, #88309, #72723, #7845, #45208, #23467, #36732, #29651, #52333, #15425, #44292, #81211, #16357, #74110, #88773, #39974, #3547, #89697, #83068, #11579, #24382, #24863, #39040, #17299, #53746, #75059, #53261, #90172, #47072, #69345, #54657, #39495, #83531, #60392, #59934, #60854, #18690, #40427, #89230, #4475, #54200, #61782, #46155, #52791, #10170, #17759, #82143, #68417, #90614, #25775, #68889, #67951, #11107, #4019, #47553, #82612, #46613, #23921, #75514, #10636, #81670, #3076, #61335, #31960, #18222, #75979, #9710, #16818, #32894, #32436, #25320, #31504, #76458, #45676, #74583, #38591, #67494, #2625, #26733, #57038, #91084, #48487, #84011, #56572, #92506, #26255, #77866, #6360, #92044, #71709, #33352, #34306, #91577, #35233, #92991, #55149, #19159, #5439, #5898, #84469, #63212, #42322, #13016, #70765, #48016, #20573, #64158, #69814, #27198, #55620, #78333, #34768, #62249, #40896, #76921, #63683, #21028, #12049, #12524, #4950, #41852, #33836, #71233, #27674, #49896, #28149, #56085, #85425, #49445, #62745, #84937, #13475, #20089, #48970, #85876, #78791, #13934, #19619, #42793, #77386, #41374, #70308, #1564, #21968, #37091, #7740, #72618, #65082, #8657, #73082, #35710, #80632, #44175, #36621, #29993, #52218, #182, #65543, #79724, #57955, #658, #50841, #29063, #66000, #87723, #16244, #30447, #80178, #59339, #7283, #6836, #29542, #88191, #81101, #36161, #45094, #1112, #37535, #86810, #93450, #14866, #58422, #43720, #15316, #66446, #23351, #15788, #87268, #51739, #44647, #64624, #22414, #51286, #28605, #8213, #58877, #57494, #22874, #73548, #86337, #21487, #50367, #79271, #14411, #43269, #72167, #12045, #4471, #92501, #62245, #5435, #70304, #27193, #76915, #26251, #56568, #90610, #48011, #83527, #56080, #92038, #25771, #77382, #5893, #91572, #71228, #32890, #33832, #91080, #34763, #27670, #54653, #18685, #4946, #34301, #84007, #62741, #41848, #12520, #63208, #47549, #20085, #63678, #69340, #26729, #55144, #77862, #84933, #61777, #40422, #76453, #48966, #20569, #11574, #40892, #33348, #41370, #69810, #70760, #13012, #49441, #85421, #55615, #84464, #78329, #19614, #48483, #13469, #42319, #36616, #7279, #72163, #64620, #8207, #72613, #35228, #80173, #43714, #36156, #29536, #51734, #93446, #65078, #79266, #57490, #177, #21483, #28600, #65537, #87262, #15783, #1106, #79719, #29987, #6832, #6355, #29057, #58871, #80627, #35706, #44641, #653, #37086, #86332, #92987, #50362, #57950, #14406, #14861, #65995, #87718, #15311, #43265, #51280, #44170, #22869, #86804, #21962, #64154, #50835, #7735, #28145, #58416, #22408, #73077, #57034, #85872, #49891, #21023, #78788, #13929, #42788, #71704, #39376, #9107, #46035, #17171, #67829, #23801, #66892, #3413, #37529, #88653, #30442, #2954, #38920, #66439, #24259, #46491, #38470, #18094, #73543, #74449, #37984, #75394, #68292, #1559, #59334, #45548, #74940, #30922, #9582, #82492, #53133, #10050, #88186, #60730, #10507, #16239, #67374, #2032, #24740, #31840, #8652, #81095, #23345, #89569, #61211, #52213, #52665, #45089, #82013, #73990, #17640, #53622, #90046, #32307, #2503, #25198, #54072, #59812, #82942, #81545, #31381, #16693, #60270, #89107, #75850, #54534, #68765, #19493, #35934, #86568, #26121, #83403, #55494, #18553, #86108, #48359, #64852, #21257, #19037, #26603, #5313, #10973, #11921, #91914, #76795, #4818, #43041, #62125, #77262, #47892, #40770, #11456, #50127, #12392, #39842, #27068, #84342, #69688, #70179, #93679, #40308, #33700, #55015, #4352, #62611, #90956, #69223, #41238, #34182, #57721, #71943, #63085, #7064, #47421, #46948, #91453, #28837, #3895, #76331, #32772, #55955, #79026, #33229 ),
 ( #14180, #83887, #61660, #90492, #25651, #51059, #87953, #59111, #16024, #65779, #15085, #45332, #79503, #36864, #72393, #44875, #80877, #14639, #66224, #88439, #80401, #60053, #21737, #22641, #79947, #23588, #81329, #43497, #7510, #87491, #23106, #72842, #51513, #30689, #1338, #51988, #36395, #8892, #16476, #888, #73777, #15548, #44419, #43945, #52455, #37770, #50613, #1803, #66675, #73326, #59589, #67151, #7970, #8437, #29771, #58650, #37316, #30220, #74233, #9352, #38237, #31167, #2284, #65308, #416, #22191, #29303, #58197, #87041, #40554, #24505, #69468, #83192, #90740, #75177, #81794, #10290, #46733, #53387, #68541, #25898, #54780, #69012, #82271, #40096, #4143, #76579, #17881, #24990, #33473, #75636, #10759, #88891, #17424, #90288, #3197, #18340, #47195, #38708, #24039, #76109, #89349, #68072, #60514, #83659, #46273, #61457, #32565, #11242, #39160, #32081, #18822, #52915, #60982, #45805, #33014, #54317, #16942, #39616, #61905, #53863, #74715, #9835, #89830, #82729, #47678, #11702, #67615, #2743, #3680, #25440, #4600, #31623, #71352, #13135, #6015, #19280, #49559, #93111, #5081, #27322, #26851, #13590, #63801, #91221, #69938, #84130, #34890, #50015, #6951, #41503, #33962, #70884, #62866, #6483, #92630, #78908, #35362, #34427, #41971, #20689, #26388, #56208, #42442, #92165, #20219, #27802, #55275, #56695, #64283, #85067, #62376, #48139, #63334, #55739, #28266, #57155, #77041, #12172, #49097, #85541, #19741, #77995, #85996, #78454, #21145, #41015, #14055, #42919, #91699, #71833, #84591, #48609, #77509, #12658, #70431, #5557, #8330, #23478, #74120, #14978, #43384, #44303, #72279, #73670, #37211, #52344, #8781, #7856, #15437, #87846, #64738, #779, #80763, #65665, #87387, #30571, #50955, #66118, #36743, #29662, #303, #37659, #1232, #93566, #15915, #73214, #58542, #58997, #81221, #29183, #22534, #43834, #86933, #51406, #79838, #58080, #30114, #22995, #45218, #59468, #51870, #88323, #36280, #35824, #80298, #16367, #28723, #65200, #57608, #44770, #66567, #22085, #86451, #72736, #1689, #21609, #50492, #79393, #14529, #7399, #2635, #54210, #83079, #90626, #31971, #39049, #47565, #60864, #24874, #9241, #67505, #10648, #17310, #32446, #61349, #52801, #38119, #90183, #9722, #82154, #74593, #68902, #38601, #75525, #46625, #3557, #53270, #31514, #32906, #67030, #24393, #59942, #25331, #39506, #88782, #18234, #39985, #45685, #67961, #60402, #47086, #68427, #2166, #16828, #31055, #75990, #25788, #23930, #46165, #89240, #17770, #75068, #11119, #4034, #54670, #61794, #10180, #82622, #83543, #81679, #3086, #18701, #89707, #53756, #71247, #91590, #13030, #77400, #48500, #40908, #78346, #48984, #11591, #56585, #20102, #12536, #5911, #28164, #69828, #41387, #55632, #33848, #70320, #26746, #4963, #41865, #63696, #85890, #6376, #56098, #35247, #76933, #76471, #5451, #64173, #57054, #12061, #21042, #70778, #13488, #62757, #69356, #84482, #34319, #19631, #84953, #42335, #93005, #85438, #63225, #27687, #20588, #40439, #92057, #27211, #4486, #77883, #34781, #33363, #92522, #49458, #62264, #91097, #26267, #55161, #84024, #19170, #48028, #29077, #21503, #15804, #79284, #22428, #87281, #44193, #195, #43283, #73564, #13951, #65095, #6850, #73097, #15332, #42807, #671, #22890, #14878, #88209, #49910, #50854, #14425, #51760, #44663, #71723, #35725, #21980, #51300, #7296, #79736, #58892, #29555, #64638, #78805, #37105, #65557, #43732, #66014, #87738, #93466, #1126, #59358, #58436, #86352, #1580, #72180, #28619, #80193, #30007, #57508, #50380, #36176, #8227, #80649, #8673, #37551, #66462, #72632, #30462, #57968, #86822, #7752, #36637, #24280, #23366, #2525, #38941, #89129, #53155, #3438, #31861, #23822, #89591, #59832, #39866, #31402, #46515, #10073, #90069, #9604, #66916, #75873, #24761, #52233, #82037, #18119, #52685, #38005, #81116, #81566, #17194, #32332, #32793, #46055, #60750, #67850, #17662, #3917, #82966, #74961, #2976, #46971, #10998, #53644, #82514, #16714, #25221, #61234, #60292, #54094, #75416, #74011, #16259, #10532, #39399, #68787, #68314, #61682, #45109, #9128, #2053, #30944, #88673, #45569, #74474, #38492, #67397, #27563, #55977, #77761, #19980, #83908, #92403, #26145, #91475, #18580, #62149, #40793, #84831, #54556, #90978, #56459, #12910, #78231, #55039, #19060, #69710, #13370, #48381, #47915, #20470, #49337, #34203, #4841, #5335, #47445, #83424, #76354, #35123, #11480, #26625, #48857, #42211, #76818, #55516, #33725, #11944, #84365, #62635, #19514, #27090, #41748, #6255, #85320, #70202, #71125, #77284, #90513, #12414, #25677, #40330, #41265, #69246, #70661, #4374, #63108, #33252, #91936, #5790, #34664, #63578, #1018, #29896, #44074, #57392, #15218, #72976, #51643, #86702, #83, #8562, #21866, #79626, #64045, #28500, #65437, #72071, #87168, #22317, #13831, #92886, #51188, #64524, #43170, #35608, #58780, #93349, #36521, #7637, #58325, #14309, #86234, #87623, #28047, #79163, #20924, #80075, #29434, #56937, #14767, #36992, #28962, #85774, #49793, #64980, #21386, #65904, #22774, #78690, #42682, #36063, #552, #50255, #57848, #8106, #43620, #80529, #71601, #15683, #44548, #6735, #50742, #7188, #73451, #72517, #66350, #44999, #59240, #9960, #25113, #75765, #16605, #73901, #45940, #9017, #75302, #38832, #53987, #10421, #9483, #17072, #89479, #1465, #2413, #82402, #67283, #89017, #32213, #52576, #67739, #38370, #31293, #1931, #39285, #2865, #30351, #17550, #74847, #68203, #46402, #30826, #3323, #61120, #82856, #60179, #24164, #37441, #53045, #81920, #88086, #59722, #31749, #45460, #60641, #24639, #81004, #23244, #53527, #37896, #74360, #66801, #89958, #88565, #18008, #46861, #52122, #81456, #23713, #16147, #68674, #26030, #61575, #34094, #70079, #3808, #55404, #77646, #69598, #49226, #10885, #11829, #69136, #12797, #70557, #32689, #90407, #76703, #77172, #62032, #40680, #19872, #84257, #48270, #25564, #91827, #41638, #47321, #4728, #4264, #55871, #12302, #39748, #18463, #54444, #41146, #92293, #83317, #83793, #76238, #19407, #11369, #48742, #5222, #27450, #5680, #33606, #62996, #26981, #40220, #62514, #84723, #91355, #26515, #34555, #54913, #63464, #56342, #85204, #33142, #20354, #90866, #18947, #47802, #21758, #14199, #7531, #29790, #42572, #43060, #57286, #35499, #71964, #93241, #71488, #14662, #65332, #87514, #72864, #57742, #7990, #78581, #78123, #79048, #36883, #58670, #13719, #22661, #72415, #79968, #64414, #71013, #28394, #35955, #6619, #86587, #15105, #28856, #51080, #7082, #13261, #42098, #64874, #86128, #43965, #65798, #6145, #35016, #50149, #50633, #21277, #93700, #87061, #79523, #43517, #63931, #436, #910, #20816, #36416, #29324, #58217, #22210, #92769, #85668, #27937, #56827, #49686, #91110, #30710, #59131, #60073, #87974, #90638, #24060, #69368, #25801, #23606, #31187, #11132, #80423, #16498, #4046, #81348, #9374, #47577, #66696, #81813, #52474, #45350, #16042, #54681, #52936, #15568, #32916, #88910, #74252, #76001, #4498, #44895, #38257, #59609, #8912, #67171, #1824, #73798, #18243, #39996, #62275, #76482, #47095, #11605, #52009, #51534, #2304, #40450, #33376, #80895, #44439, #68915, #83555, #37789, #73345, #88459, #61806, #18714, #8456, #37337, #66243 ),
 ( #1358, #30241, #23126, #5462, #57065, #70788, #76945, #84035, #5923, #20115, #85903, #41877, #71260, #13964, #48997, #56111, #64651, #77896, #34793, #26279, #84496, #27699, #34332, #49469, #78359, #69840, #55174, #13499, #26758, #63238, #91602, #21055, #55643, #92533, #63708, #20599, #70333, #19642, #49922, #19180, #41399, #12072, #42347, #85451, #48040, #56597, #93017, #84964, #40920, #4974, #27223, #48510, #28175, #78819, #33860, #62770, #92069, #6388, #77411, #13040, #35259, #64185, #42822, #12549, #71737, #6863, #35738, #58453, #57986, #44680, #1144, #28633, #7312, #21518, #66031, #81134, #38025, #72647, #36191, #8242, #65110, #37571, #30025, #16278, #66481, #65574, #73115, #51778, #57522, #87297, #73582, #29572, #51316, #88228, #14893, #58908, #688, #22443, #86839, #1598, #87754, #86367, #8691, #37122, #80208, #22907, #45129, #21997, #15348, #7769, #50869, #44208, #43747, #79751, #80667, #15823, #9147, #23384, #30481, #52253, #213, #93480, #59376, #74030, #50396, #29093, #79301, #14441, #43298, #36653, #72195, #53177, #24782, #2545, #46534, #3938, #32812, #46992, #60313, #18138, #11500, #23840, #59851, #66934, #54115, #82533, #2995, #82988, #75894, #88692, #11018, #76374, #75436, #9625, #18602, #89151, #81587, #68336, #39888, #30963, #2072, #16735, #39419, #68809, #3459, #10554, #32354, #60771, #83447, #67416, #31424, #61253, #52706, #67872, #45590, #46074, #17682, #38960, #31881, #61702, #90089, #24300, #25241, #38512, #47467, #74980, #90534, #53664, #25694, #82056, #74493, #54576, #17213, #10092, #89611, #27584, #47935, #91000, #4395, #76838, #84386, #70680, #13388, #19535, #91957, #70221, #20001, #42231, #56481, #48401, #5356, #85339, #20490, #77304, #34222, #11965, #34684, #5810, #91492, #63598, #63128, #62169, #69266, #27112, #12436, #92422, #55996, #48879, #33272, #84851, #49356, #26169, #26647, #78250, #55060, #40813, #40349, #83929, #19081, #69730, #4863, #77782, #33746, #12930, #41770, #55537, #62658, #41286, #90374, #88983, #31714, #90830, #18426, #18911, #89442, #60606, #75268, #47766, #82818, #2832, #54875, #83755, #68635, #10382, #39711, #53009, #24131, #81884, #76664, #24601, #61079, #39250, #82365, #25077, #46366, #53489, #61541, #47285, #40641, #25989, #10847, #11791, #17515, #31257, #32178, #69561, #60145, #68165, #17039, #25529, #33105, #3285, #45905, #89921, #17970, #53951, #3768, #61994, #74811, #11331, #46822, #76202, #40182, #9926, #75725, #32653, #38800, #54409, #83281, #67703, #69101, #4228, #12756, #27901, #56789, #48230, #4689, #85631, #5178, #41596, #70037, #64379, #34053, #70975, #42061, #92729, #48701, #91789, #28356, #62474, #19833, #55366, #20777, #63893, #91316, #49188, #71445, #63427, #43023, #33564, #5645, #62955, #6582, #93204, #26477, #84218, #70519, #6108, #55828, #34520, #42534, #78082, #34979, #77132, #49650, #35460, #41106, #92256, #26940, #78544, #57247, #12263, #84684, #27413, #86090, #21240, #56301, #85167, #20318, #13226, #50109, #79004, #14159, #88419, #16004, #43928, #51495, #30202, #7048, #36845, #23085, #7950, #29751, #66657, #87023, #8419, #72824, #65762, #36377, #73759, #44400, #35917, #51966, #15524, #872, #1320, #59093, #93659, #80383, #8871, #64835, #79930, #37749, #57703, #72375, #71926, #1784, #37298, #87934, #80857, #65291, #30667, #7492, #58632, #28820, #43479, #22174, #66204, #86546, #395, #59570, #44856, #23569, #29285, #58181, #51042, #52436, #87473, #15066, #81311, #16457, #73308, #22621, #21717, #50592, #79486, #14621, #83637, #2265, #38216, #45309, #32546, #60957, #75158, #61438, #54298, #67131, #90269, #54760, #24970, #81773, #90718, #67595, #60034, #46713, #25420, #9333, #74214, #88871, #17862, #83170, #75616, #53845, #10740, #39140, #61886, #45782, #74694, #82711, #31147, #46254, #24020, #24485, #89809, #17406, #10270, #18321, #39597, #9816, #68520, #16923, #25878, #53365, #3657, #32062, #47177, #31604, #52894, #4123, #76087, #38689, #68051, #40076, #2724, #60493, #89330, #82251, #3178, #11221, #68993, #32995, #56188, #34408, #13116, #93094, #78436, #48590, #63315, #13572, #42422, #19719, #92146, #77022, #85524, #27782, #91681, #49541, #27301, #69449, #76560, #85048, #12635, #71334, #20197, #4579, #41952, #77974, #11683, #49076, #20669, #77490, #57135, #18801, #41481, #12151, #6464, #35339, #40533, #33454, #84572, #70865, #69919, #70412, #56676, #5996, #34869, #62356, #63782, #64265, #55256, #5537, #40996, #92611, #28248, #47659, #26367, #91198, #84111, #19261, #48119, #26832, #5058, #33942, #62847, #55720, #58525, #8765, #30097, #58062, #65646, #44287, #21127, #50937, #37196, #22069, #43818, #80746, #7382, #22518, #86915, #79821, #50472, #87829, #87368, #49995, #66103, #29645, #14962, #15419, #37644, #79376, #72717, #65183, #43368, #7840, #36262, #14512, #51389, #73194, #1674, #15898, #761, #44754, #86434, #85977, #36727, #73655, #66552, #21593, #30556, #80280, #22980, #72264, #78890, #286, #8313, #29166, #1215, #51854, #14037, #58981, #42899, #71812, #6933, #35806, #64720, #93546, #28705, #57590, #75055, #59454, #23915, #60849, #67490, #82608, #17755, #9224, #88305, #46608, #59930, #38587, #31040, #25316, #88769, #31956, #3071, #53742, #9706, #52787, #83064, #23463, #74578, #67948, #81665, #89692, #2150, #75974, #2621, #75510, #46151, #32431, #45670, #38105, #18218, #24858, #52329, #24377, #54195, #16813, #74105, #81206, #31499, #60387, #68413, #68884, #89226, #10632, #10166, #39490, #39968, #47068, #53256, #39035, #11103, #4014, #82138, #3542, #17295, #61330, #90168, #16352, #45202, #67015, #51904, #30144, #16860, #59973, #3116, #45717, #82188, #80796, #38631, #60893, #15944, #74153, #89743, #73701, #1718, #1262, #24904, #60432, #75556, #8810, #59506, #30603, #52375, #67066, #81250, #16397, #38150, #2201, #31085, #88811, #23958, #52834, #67534, #4063, #68932, #18735, #56129, #91131, #11154, #63255, #92086, #76962, #47596, #48058, #61377, #3591, #90210, #77916, #25359, #32480, #39534, #26775, #55194, #69385, #55661, #48528, #54239, #84513, #49019, #19198, #76022, #84982, #61825, #83109, #40938, #19660, #18260, #68457, #47113, #12091, #77429, #69858, #4994, #33879, #33394, #20135, #40015, #32933, #62787, #90658, #40468, #25818, #76498, #84051, #11622, #4518, #12571, #41420, #54698, #70352, #62293, #91620, #26301, #5478, #34348, #27242, #14458, #228, #70806, #41894, #27719, #79320, #29108, #43315, #86382, #72211, #6881, #30857, #13514, #42364, #21533, #92550, #13980, #13058, #85919, #28648, #78834, #42840, #86859, #50415, #71276, #7327, #49485, #59751, #21070, #36207, #93495, #81032, #93035, #56617, #66826, #65126, #5940, #71756, #9044, #6403, #85468, #34812, #35277, #35754, #22014, #23740, #64667, #58004, #57539, #50884, #88591, #73927, #16176, #45028, #37922, #1965, #52603, #63725, #64205, #20615, #78375, #49940, #28191, #57080, #38402, #45486, #32241, #75331, #18489, #3350, #39780, #9514, #61149, #47354, #74385, #89505, #76270, #67311, #81946, #81484, #11396, #46889, #68704, #10911, #74876, #83343, #17104, #82429, #2441, #53071, #31776, #75790, #31319, #45970, #40248, #3834, #69164, #9986, #38859, #60669, #4291, #39312, #67765, #33169, #62060, #25138, #24671, #89984, #60206 ),
 ( #89044, #2892, #53557, #32716, #24194, #17579, #90894, #61601, #26058, #46428, #10446, #68230, #16632, #54014, #82881, #18036, #90434, #25590, #54474, #63495, #76733, #18979, #11860, #93274, #40709, #47831, #54946, #42130, #70586, #84752, #71046, #63963, #69629, #6180, #64448, #34588, #91390, #6656, #77200, #4757, #56373, #35048, #33637, #83825, #62547, #27482, #92804, #85240, #92326, #20388, #48771, #71521, #55433, #84285, #49260, #26545, #55898, #19435, #34122, #5713, #27011, #19900, #27970, #78154, #48299, #13292, #12330, #35534, #63026, #56860, #41668, #85702, #41174, #70115, #13758, #20847, #5253, #77678, #49718, #91857, #12830, #78613, #42606, #29361, #37367, #37822, #472, #65835, #44002, #22693, #8944, #88010, #58253, #72899, #23163, #52047, #87096, #8024, #86621, #1390, #66276, #7563, #59164, #36920, #79081, #86159, #943, #22246, #80931, #29821, #80454, #50184, #58703, #43093, #87546, #15600, #51568, #44473, #73379, #51116, #44929, #28887, #57776, #8489, #14234, #80002, #28427, #36449, #30273, #15140, #16076, #73830, #66729, #21792, #57319, #64906, #21312, #65364, #71998, #7117, #35986, #14694, #7, #50667, #79553, #43549, #72445, #90337, #2341, #16530, #59648, #31220, #2792, #10811, #11294, #67666, #39210, #17476, #89881, #76161, #61505, #31674, #46327, #25492, #54370, #60566, #75230, #60105, #68595, #39672, #74769, #32615, #10344, #52506, #88493, #68124, #89404, #83244, #3248, #53913, #23640, #32139, #18391, #81382, #9887, #47249, #45382, #88945, #1856, #40147, #61036, #82781, #25041, #24092, #3731, #52969, #24558, #74284, #67208, #45862, #17933, #9408, #81846, #30745, #46784, #38293, #16996, #38762, #53443, #82326, #75685, #40606, #92686, #27855, #12713, #48190, #77565, #90792, #33067, #25952, #13641, #54833, #61957, #69063, #56262, #84643, #5134, #85121, #78044, #83713, #20273, #78503, #48663, #11753, #20737, #91273, #18874, #70478, #49148, #47730, #4192, #34939, #4652, #41555, #5606, #63386, #19328, #62432, #56747, #76630, #84180, #69520, #92217, #34480, #33526, #19794, #42019, #34013, #26439, #55330, #69994, #77092, #70935, #63853, #12222, #41069, #62915, #27372, #91751, #26902, #13185, #6066, #85590, #55791, #49607, #73266, #78961, #7450, #7002, #87433, #43886, #71406, #50065, #64335, #15027, #30162, #80812, #21668, #14112, #51001, #42975, #80343, #72782, #59044, #15485, #14578, #22133, #829, #6538, #36332, #22579, #72330, #352, #37258, #57657, #7907, #43434, #65246, #35875, #44356, #36797, #35415, #51454, #79886, #29239, #65717, #87892, #64791, #58134, #50545, #93616, #86980, #86505, #28774, #29711, #58593, #51922, #66164, #8378, #1279, #71881, #42492, #23044, #93162, #28315, #79442, #57204, #86045, #21194, #2219, #8829, #31103, #67552, #45268, #89287, #46668, #75572, #89760, #9288, #60914, #24922, #3610, #38648, #45737, #54255, #2681, #31560, #15961, #74171, #17360, #23978, #39093, #68006, #59525, #44815, #3135, #16415, #88829, #81270, #38170, #46212, #32015, #25375, #10694, #24440, #39551, #67086, #73718, #16878, #68474, #61394, #59990, #90225, #10226, #17815, #52852, #37708, #81730, #60452, #74647, #53321, #32496, #66614, #53798, #9774, #82667, #1736, #30624, #82206, #75116, #88374, #23524, #52393, #83125, #47613, #84527, #91151, #12589, #41435, #32950, #18276, #70367, #83592, #62310, #54714, #49033, #18755, #55677, #26791, #77444, #33411, #76516, #13072, #47130, #4535, #40033, #5492, #48543, #76043, #33895, #56144, #48074, #27735, #11172, #84066, #11639, #84996, #77929, #68949, #4080, #55212, #19675, #40486, #19216, #92102, #62802, #34365, #61843, #63270, #20152, #25835, #76978, #69402, #27257, #41908, #90675, #26317, #12107, #70821, #5953, #40953, #69874, #5013, #91637, #34826, #63738, #92564, #73149, #718, #28663, #36220, #14923, #85482, #21547, #7797, #86395, #14471, #51347, #71771, #86874, #57550, #50432, #21084, #58482, #29122, #20629, #36682, #241, #79336, #79780, #8273, #49955, #43328, #35768, #13994, #72226, #6893, #65605, #44238, #7340, #65140, #1173, #58019, #22028, #56632, #78847, #50897, #64681, #43776, #72678, #6417, #49499, #29604, #57094, #93507, #28206, #22474, #85934, #87326, #80239, #15376, #37153, #42856, #66061, #78389, #13529, #42378, #71291, #35293, #64219, #93050, #3026, #88724, #68365, #30055, #30997, #88263, #31912, #89643, #51808, #87787, #2107, #2576, #81165, #59884, #38990, #74526, #67448, #80702, #17247, #60804, #66510, #23872, #23420, #75012, #31454, #58936, #37600, #15853, #60343, #17713, #22937, #9180, #1630, #38545, #30512, #67903, #89180, #46566, #24814, #52738, #9661, #82088, #44711, #81620, #10124, #16769, #45623, #53697, #45161, #24332, #53209, #46107, #52285, #82565, #75465, #73612, #10586, #39449, #8723, #59408, #16309, #74060, #38058, #66967, #54609, #91032, #18637, #61735, #33782, #84421, #12966, #91994, #76872, #27147, #3971, #3494, #4426, #56033, #48916, #32845, #77817, #91527, #5392, #83480, #90121, #47504, #55097, #90567, #11998, #34257, #63163, #77339, #25725, #48435, #19113, #33304, #19569, #12473, #25273, #41321, #41805, #40847, #39924, #32387, #76411, #18171, #4897, #70258, #61287, #54150, #47024, #69766, #84887, #62697, #26683, #55573, #26202, #20038, #11533, #40380, #83019, #75927, #62202, #11053, #69297, #47968, #83964, #68843, #50792, #79220, #71183, #43222, #13425, #87218, #78742, #132, #57447, #43673, #56990, #20527, #29492, #72123, #5847, #35664, #65490, #6312, #85378, #34719, #35180, #71655, #79676, #80127, #42740, #14363, #86288, #65032, #51239, #36575, #6788, #21441, #607, #58375, #64579, #50315, #64103, #72568, #14818, #49846, #7690, #7239, #27621, #63633, #36115, #93404, #22365, #29015, #57900, #92458, #86756, #15266, #56519, #13886, #70716, #49396, #92943, #78287, #42270, #21918, #28103, #85828, #20979, #28556, #73501, #45048, #65955, #15736, #88139, #9538, #8158, #44598, #10008, #31340, #31796, #8613, #37489, #23297, #60690, #1986, #66399, #67786, #2912, #81505, #52171, #52623, #1066, #37041, #29945, #82452, #58830, #87675, #44126, #60227, #1515, #81053, #38423, #22826, #30401, #38879, #89066, #89530, #59293, #16196, #73949, #24694, #30877, #9064, #53577, #73030, #16652, #37942, #45506, #51694, #80583, #66851, #59771, #88612, #23759, #74408, #24216, #67332, #2464, #53091, #81970, #17126, #45992, #74897, #90915, #54034, #64351, #39802, #32263, #18999, #6079, #75352, #46450, #61169, #83846, #34953, #47852, #26081, #76754, #11417, #35429, #18057, #46909, #54970, #3375, #18513, #17600, #90455, #33192, #83363, #47377, #92699, #13197, #75810, #42033, #82901, #93177, #25612, #70947, #4314, #85603, #3854, #90005, #71418, #63865, #10467, #76291, #13654, #10934, #25160, #39333, #68724, #40268, #27869, #28329, #69185, #56762, #62082, #20750, #57219, #78517, #49621, #42506, #6550, #68251, #32734, #61623, #54495, #59060, #1294, #65260, #23059, #36811, #42991, #50079, #65732, #79901, #51937, #7920, #44369, #14126, #843, #80827, #78974, #366, #15978, #71897, #86517, #86059, #44830, #51468, #73280, #15498, #79456, #87908, #21682, #86994, #7017, #50559, #35888, #64806, #14591, #22146, #30176, #1754, #58148, #29724, #58606, #80357, #66629, #73733, #51014, #87447, #8845, #37723 ),
 ( #15039, #22593, #43448, #43899, #30641, #8393, #37271, #93630, #66177, #21209, #28787, #72796, #72345, #57674, #7463, #36346, #29252, #81286, #32035, #47150, #4095, #38664, #67102, #68025, #2236, #3626, #60930, #76059, #32514, #31579, #39112, #17835, #88390, #24459, #10712, #89303, #17377, #54271, #74665, #89777, #60468, #53338, #23995, #61410, #24940, #23541, #39569, #3152, #82223, #82685, #11188, #52868, #46229, #67568, #16897, #75133, #9789, #81747, #53817, #46687, #68965, #83141, #75589, #18292, #60006, #59540, #10243, #40048, #52411, #88846, #16432, #68491, #90242, #45755, #45284, #2697, #25391, #74187, #9306, #38188, #31120, #13088, #26336, #77944, #41926, #20645, #55693, #77463, #83610, #90690, #12606, #26807, #63754, #48560, #85017, #54732, #41451, #92584, #25850, #40969, #27753, #18771, #33426, #32966, #56648, #92119, #20169, #56160, #55229, #34843, #62330, #33911, #47629, #4552, #76995, #27273, #76533, #91170, #85498, #49049, #49515, #84084, #19234, #12124, #78407, #84544, #48091, #13546, #42394, #70383, #69892, #5511, #11655, #40502, #69421, #71306, #5031, #62820, #61859, #70837, #34381, #91654, #5969, #19691, #63286, #22489, #15870, #79794, #42871, #51824, #28679, #21101, #7810, #87340, #64236, #35311, #49969, #72691, #51362, #36700, #14936, #65621, #256, #22950, #6906, #35781, #43791, #85949, #7353, #6436, #79349, #22041, #72239, #36235, #80253, #731, #64694, #29617, #71784, #80717, #14484, #58495, #86887, #73167, #86408, #78860, #58953, #15389, #93066, #65153, #1187, #93520, #14011, #28221, #57565, #29139, #44256, #44726, #58034, #8286, #50910, #37166, #57109, #66075, #30068, #87801, #21563, #50447, #43342, #38559, #45174, #3042, #39004, #59898, #31925, #23886, #52754, #10138, #2590, #16323, #60358, #52301, #82579, #88740, #82105, #9677, #60817, #66984, #88278, #53712, #89195, #8738, #81636, #89660, #81178, #30525, #37615, #74076, #16783, #67918, #75479, #45637, #31470, #67461, #53223, #10604, #24829, #74546, #24348, #17726, #46581, #17264, #46122, #9195, #73626, #66526, #75025, #1645, #59427, #38073, #2122, #23433, #31011, #1486, #80096, #22792, #86255, #44093, #30369, #28521, #72538, #59258, #50279, #65002, #64545, #88106, #29915, #51661, #87644, #57869, #66368, #104, #65457, #21406, #36083, #14787, #58799, #57416, #28983, #23264, #80548, #52142, #86725, #21889, #43640, #81022, #22336, #50761, #16166, #45018, #8127, #7657, #72998, #79187, #14331, #43191, #9036, #72091, #7208, #93371, #15705, #15237, #574, #44566, #73469, #79645, #8581, #73919, #37011, #36542, #29458, #58346, #87187, #65925, #37459, #51207, #1037, #52594, #10438, #25130, #39304, #17569, #3341, #31768, #54464, #38391, #67303, #46420, #23731, #38849, #37914, #17093, #53548, #68694, #3825, #18026, #31311, #82873, #46880, #25581, #60660, #67757, #76259, #89497, #82421, #66818, #2431, #68221, #45961, #61140, #89976, #81475, #1951, #54004, #60197, #74866, #9503, #32706, #89035, #32232, #75321, #75782, #81938, #24185, #61592, #30848, #53063, #88583, #10902, #39769, #59741, #90424, #83334, #2883, #16624, #45478, #24660, #9978, #18480, #47342, #74377, #69154, #77191, #77666, #62535, #41164, #20376, #55889, #48761, #62051, #92315, #42117, #47820, #70101, #69618, #56362, #12818, #40239, #18967, #33160, #41658, #92789, #49704, #84275, #76722, #19890, #11848, #49247, #70575, #27957, #78142, #12320, #84743, #63484, #4282, #5242, #85225, #34113, #63015, #6167, #26534, #5700, #91846, #27001, #4746, #13280, #34575, #90885, #71033, #27469, #35036, #63950, #56847, #33626, #85688, #19426, #91376, #20835, #55422, #48288, #11387, #26048, #54934, #83814, #40698, #73361, #79067, #78600, #79541, #37353, #30257, #14219, #59149, #72884, #80439, #64893, #71507, #26508, #36435, #43079, #58237, #65818, #79987, #87081, #43987, #72433, #1375, #71984, #7102, #22230, #64434, #14680, #13743, #57761, #457, #50653, #43536, #58687, #51100, #35973, #15124, #21298, #87993, #86607, #8009, #65350, #51551, #28874, #28414, #66260, #36901, #42592, #7550, #8473, #21777, #93260, #6640, #29344, #926, #87530, #23146, #29806, #22678, #15584, #44455, #35520, #57305, #86147, #50170, #17918, #75669, #52952, #2776, #16515, #25025, #61019, #31204, #82765, #31657, #8928, #16059, #60548, #45845, #46768, #67650, #10328, #73815, #89387, #10794, #44912, #60089, #39654, #37806, #52490, #52029, #68578, #17459, #39195, #75214, #45366, #53897, #81365, #81830, #66713, #23623, #2324, #46309, #1841, #74269, #3714, #68107, #32599, #9392, #38276, #88928, #61489, #9870, #67189, #90321, #80914, #24541, #24076, #53425, #30728, #59629, #88476, #16980, #74750, #38746, #82309, #3232, #32123, #89865, #12697, #34461, #18374, #41536, #34921, #5118, #61939, #70916, #47714, #40130, #26887, #70462, #83228, #54355, #69047, #91734, #47232, #84164, #5589, #55312, #77075, #20254, #40590, #55774, #26421, #91257, #83695, #27355, #84627, #76143, #63369, #62898, #19312, #48646, #6049, #18856, #48174, #4635, #76614, #12206, #69504, #11737, #19775, #92199, #63835, #49130, #33995, #78026, #25935, #25475, #41051, #13166, #11277, #54817, #4176, #77546, #56243, #33509, #33049, #62415, #69977, #85104, #42002, #90776, #29691, #72765, #86028, #43868, #7888, #80325, #21650, #28757, #37242, #50527, #14560, #92666, #57187, #334, #6984, #22115, #50984, #42475, #27838, #79869, #93142, #71863, #64317, #58575, #28297, #65229, #36313, #86962, #42957, #21177, #22562, #56727, #14093, #49590, #15009, #58117, #85573, #43417, #65697, #57640, #20720, #78486, #93599, #50046, #811, #87415, #13622, #71387, #64774, #29219, #78943, #86485, #36778, #72312, #51436, #6519, #15466, #44338, #35397, #79425, #35857, #73248, #8359, #7433, #18241, #32456, #76942, #92066, #48994, #83552, #47093, #19177, #75998, #48507, #12069, #27220, #77408, #76479, #84032, #62767, #33857, #69837, #68434, #55171, #12546, #69365, #10657, #39513, #11602, #68912, #41396, #70330, #61356, #3566, #40447, #40916, #61803, #4495, #19639, #48037, #4971, #90190, #91599, #5459, #11129, #33373, #4043, #55640, #26755, #25338, #39993, #54218, #84493, #56107, #83087, #18711, #32913, #34329, #90635, #63235, #84961, #20112, #25797, #62272, #54678, #47574, #91107, #26276, #29090, #13961, #35735, #72644, #93014, #14438, #78815, #49919, #42345, #79748, #50393, #13037, #57983, #21515, #42819, #7309, #29569, #71256, #71734, #57062, #35256, #6860, #28172, #6385, #43295, #65107, #87294, #7765, #57519, #36650, #78356, #77893, #64648, #65571, #58449, #13496, #22440, #72192, #14890, #64182, #70785, #85900, #93477, #21052, #86363, #43744, #685, #86836, #28630, #21993, #50866, #41874, #79298, #36188, #5920, #209, #34790, #63705, #92530, #27696, #56594, #85448, #20596, #49466, #51313, #38509, #51775, #30477, #22903, #17210, #80664, #23837, #88689, #45586, #1595, #44677, #74977, #15344, #66478, #8239, #67413, #44205, #80205, #66028, #52703, #2542, #81584, #30960, #16732, #45126, #67869, #15820, #73579, #59848, #37119, #52250, #73112, #59373, #66931, #23381, #81131, #31421, #74490, #8688, #9622, #87751, #2992, #88225, #60310, #38021, #24297, #37567, #1140, #10089, #89148, #30022, #16275, #46071, #74027, #58905, #9144, #2069, #53174 ),
 ( #82053, #38957, #31878, #60767, #89608, #24778, #25690, #82984, #26643, #84382, #46531, #82530, #90530, #90995, #75889, #54572, #33741, #69262, #62165, #75433, #11961, #55533, #61250, #83443, #18134, #69726, #26164, #53661, #32351, #10551, #55056, #12431, #63124, #3934, #90085, #33268, #25237, #62654, #83925, #41281, #91489, #18597, #4391, #76834, #17679, #47463, #4858, #76370, #11496, #19531, #39884, #19077, #40345, #47931, #46988, #48397, #40809, #39416, #77300, #70218, #5352, #34218, #54111, #68333, #11014, #3456, #68805, #32808, #61698, #19996, #64539, #79640, #36537, #71141, #5806, #6751, #34680, #36078, #93365, #14782, #64996, #64061, #71617, #50272, #27108, #56952, #43185, #28062, #49809, #86719, #13384, #28515, #92903, #85789, #56476, #99, #57409, #55992, #72087, #35624, #20940, #21400, #43635, #85335, #78705, #6270, #49352, #13847, #42227, #20486, #86249, #79180, #7652, #21884, #14325, #50756, #92418, #91953, #42699, #72533, #84847, #27579, #48874, #7203, #28978, #78247, #77778, #35138, #57863, #12925, #41766, #70677, #63594, #45474, #58795, #16620, #74374, #53059, #88101, #1480, #9974, #23260, #81018, #65452, #29911, #66815, #73465, #88579, #23727, #15233, #568, #52590, #65921, #44562, #37008, #31307, #1033, #37910, #9032, #59737, #15700, #87639, #89031, #29453, #80544, #22332, #81471, #30843, #58341, #16162, #38386, #30365, #87183, #51203, #66364, #22788, #67299, #60193, #80091, #44089, #37455, #1946, #51657, #59254, #9498, #45014, #2427, #72993, #24180, #81934, #52138, #73915, #8577, #17088, #45956, #74862, #8122, #24655, #38846, #67753, #82417, #53543, #75317, #17565, #46416, #2879, #31764, #60656, #89493, #42332, #66339, #20099, #34778, #34316, #1453, #93463, #22760, #57505, #27684, #37430, #63693, #35243, #56095, #5908, #78343, #28616, #92054, #92518, #30339, #51631, #23231, #56582, #85435, #13485, #52111, #85887, #20585, #59229, #88075, #71720, #71243, #42804, #84949, #27208, #48981, #73889, #77879, #13026, #63222, #80517, #49907, #64170, #15670, #44537, #41862, #73440, #44988, #13947, #70775, #80994, #49455, #6372, #35721, #8550, #93002, #28160, #57051, #6847, #16136, #64635, #86349, #21039, #78802, #25555, #9472, #38358, #17540, #88554, #9950, #9006, #81910, #24629, #74837, #38822, #82846, #46392, #67272, #75292, #45449, #54435, #17062, #32202, #89468, #75754, #89006, #52565, #61565, #10411, #37885, #67729, #3798, #2402, #23702, #66790, #31282, #2856, #17998, #18453, #31738, #39275, #53516, #3313, #83308, #68662, #60631, #82392, #68193, #61109, #1920, #89948, #53977, #25103, #46851, #32679, #24154, #10875, #39738, #90398, #60168, #47312, #30814, #59711, #81445, #16593, #74349, #53034, #45928, #40671, #12293, #55395, #33597, #70071, #91345, #69589, #12789, #63455, #85660, #71005, #55863, #6136, #76694, #76228, #77163, #35008, #27928, #11820, #56818, #70549, #78114, #62505, #69127, #26505, #34085, #4719, #84715, #13253, #42090, #56334, #84247, #27442, #85196, #63923, #5212, #41138, #20807, #62988, #91819, #11358, #19398, #77638, #48261, #5672, #34547, #26021, #40211, #92285, #26972, #19864, #47792, #92761, #48734, #41629, #20346, #49218, #4255, #33133, #62023, #90857, #54904, #83783, #18937, #15098, #13711, #428, #22653, #14653, #87967, #49678, #50625, #14191, #51526, #15560, #71479, #42563, #21748, #22203, #7074, #79515, #58662, #29315, #87054, #6611, #36876, #80415, #86120, #43509, #43052, #901, #51073, #78573, #57278, #35491, #79961, #37327, #64406, #28848, #21269, #58209, #50141, #87506, #43958, #66235, #44431, #72407, #79039, #93233, #72857, #1350, #28386, #57734, #71956, #7982, #35947, #73337, #65791, #30233, #8448, #7523, #29783, #59123, #64866, #36408, #93692, #65323, #86579, #17893, #38250, #53399, #24052, #88902, #81340, #25003, #89360, #52001, #3208, #60524, #52926, #46285, #68554, #16488, #81805, #2296, #74244, #16954, #67163, #45343, #82284, #10302, #32576, #46746, #2753, #75647, #52466, #23118, #45819, #10770, #3691, #9366, #61469, #17435, #53874, #31179, #16035, #60064, #74725, #9846, #31634, #82740, #39630, #32094, #38719, #68083, #60996, #80887, #67625, #24518, #44886, #75189, #39172, #73788, #89841, #8904, #37781, #66688, #1816, #30702, #59601, #88451, #90751, #69479, #61915, #56219, #25909, #62875, #33971, #84602, #40565, #83671, #20230, #54330, #11712, #47209, #19752, #55749, #83204, #41024, #63344, #55286, #34899, #90299, #91233, #54792, #92176, #85079, #18351, #76120, #62390, #91709, #47688, #26398, #5567, #69950, #26861, #11252, #77520, #27332, #33024, #84140, #18833, #41514, #48619, #25451, #76590, #40107, #12672, #70440, #69022, #4154, #4610, #34438, #49107, #78004, #5092, #13144, #19289, #41980, #33484, #48148, #70893, #77052, #12181, #6025, #42931, #79401, #35833, #64749, #43844, #72286, #64293, #36288, #6493, #80306, #71840, #86941, #50503, #36753, #50024, #13599, #22541, #65207, #92642, #28733, #58550, #93119, #78463, #27814, #28275, #93575, #72743, #73226, #57617, #7408, #14537, #58091, #44314, #29669, #86460, #43392, #87394, #51414, #21621, #311, #57165, #65675, #7864, #6960, #787, #29194, #20698, #56704, #22093, #50963, #15445, #79846, #14986, #85551, #8338, #63810, #49568, #42451, #71363, #35374, #86005, #21154, #78917, #14066, #24401, #60410, #30580, #39056, #66576, #38127, #59006, #8789, #81229, #2644, #1241, #37668, #3094, #53280, #24882, #1697, #59481, #16376, #53763, #88790, #88334, #60871, #89718, #74605, #45226, #45694, #87854, #30123, #23003, #75533, #51881, #80774, #37219, #82164, #52810, #67040, #17321, #46172, #15924, #75076, #46632, #16838, #73678, #82629, #23486, #9734, #38611, #31522, #74130, #52353, #17778, #44778, #9249, #2177, #89249, #10187, #31063, #81689, #67968, #59951, #66126, #23938, #67514, #31978, #67631, #31640, #87512, #29789, #37787, #38256, #23124, #1822, #74731, #16495, #9372, #22659, #52933, #2759, #8454, #30708, #30239, #16960, #67169, #908, #73343, #51532, #2302, #53405, #10308, #44893, #37334, #74250, #66241, #9852, #31185, #82290, #38725, #66694, #45348, #24058, #58668, #59607, #45825, #88457, #23604, #60530, #80893, #60071, #52472, #81346, #59129, #89367, #88908, #80421, #24524, #81811, #17441, #46291, #75195, #87973, #65797, #73795, #52007, #15566, #16040, #8910, #44437, #1356, #48625, #33979, #18840, #62882, #39637, #39178, #40113, #91716, #84609, #68561, #19758, #33491, #41031, #25457, #32102, #54336, #90758, #3697, #47696, #69958, #5099, #19296, #32582, #84147, #48155, #26869, #61922, #69028, #77527, #25916, #54799, #68089, #61475, #40572, #47216, #62398, #91240, #82746, #3214, #26405, #83210, #18357, #10776, #55756, #75653, #4160, #76126, #77059, #4617, #61002, #46752, #89847, #55293, #25009, #53880, #11259, #33031, #76597, #83678, #12188, #17899, #30476, #51774, #79747, #87293, #66027, #42818, #72643, #58904, #43743, #65570, #8687, #29089, #44204, #14889, #7764, #72191, #15819, #80204, #71732, #87750, #51312, #36649, #37118, #59372, #7308, #683, #86834, #65106, #29568, #57982, #36187, #73111, #1139, #23380, #37566, #22439, #66477, #14437, #12678, #58448, #1594, #88224, #43294, #52249, #8238, #44676, #208, #6859, #21992, #15343, #50865, #30021, #73578 ),
 ( #22902, #80663, #35734, #64647, #93476, #28629, #57518, #86362, #21514, #50392, #79296, #18133, #2991, #39415, #9143, #60766, #46987, #45125, #89147, #75888, #66930, #81583, #81130, #11013, #46530, #68332, #10550, #74489, #82983, #16731, #82052, #38020, #52702, #31420, #45585, #9621, #60309, #3933, #38956, #38508, #39883, #68804, #24777, #24296, #89607, #2068, #74026, #30959, #25689, #59847, #88688, #16274, #3455, #31877, #17209, #32350, #90084, #23836, #61249, #90529, #53660, #67412, #32807, #2541, #53173, #82529, #25236, #46070, #74976, #10088, #17678, #54110, #75432, #61697, #67868, #48396, #71140, #55055, #83924, #63123, #40344, #55532, #54571, #33740, #70217, #26642, #84381, #34679, #91952, #19076, #27107, #90994, #6269, #62653, #77777, #41280, #27578, #40808, #4390, #13383, #55991, #83442, #19530, #49351, #47930, #69261, #18596, #76833, #77299, #63593, #64060, #12430, #84846, #5351, #48873, #35137, #20485, #34217, #19995, #78246, #42226, #12924, #41765, #11960, #56475, #92417, #91488, #85334, #70676, #11495, #47462, #5805, #92902, #76369, #33267, #62164, #26163, #69725, #4857, #85788, #36077, #58794, #13846, #28514, #28061, #87638, #87182, #15232, #51202, #21399, #29910, #57408, #28977, #49808, #93364, #72086, #22331, #20939, #86248, #22787, #44088, #15699, #29452, #72992, #78704, #56951, #42698, #567, #8121, #58340, #7651, #80090, #21883, #44561, #50271, #79179, #36536, #71616, #57862, #6750, #7202, #43634, #98, #86718, #37007, #65451, #14324, #65920, #64538, #73464, #64995, #1032, #14781, #51656, #43184, #35623, #80543, #8576, #50755, #79639, #37454, #72532, #66363, #59253, #1945, #2426, #10434, #10898, #67298, #38845, #17087, #89492, #75778, #61135, #31306, #45955, #89972, #25126, #60192, #74861, #59736, #68217, #39299, #74373, #32227, #9973, #52137, #88100, #67752, #89030, #54000, #2878, #53542, #23259, #31763, #82869, #81017, #9497, #18022, #16161, #30842, #1479, #46875, #60655, #82416, #24654, #88578, #3337, #23726, #24179, #45013, #66814, #45473, #17564, #73914, #52589, #39764, #46415, #30364, #81470, #16619, #38385, #9031, #53058, #81933, #37909, #75316, #12315, #47815, #77186, #90420, #32702, #25577, #13275, #54459, #61588, #68689, #55884, #84270, #4741, #84737, #77661, #83330, #19885, #78137, #48283, #11383, #20371, #90880, #18476, #4277, #41159, #5695, #34570, #48756, #62046, #12813, #41653, #56356, #91370, #33621, #3821, #26529, #19421, #47337, #33155, #70095, #76717, #91841, #26996, #76254, #40234, #70570, #69149, #11843, #26043, #63479, #54928, #5236, #34108, #63010, #18962, #83809, #92309, #40693, #69612, #62529, #27464, #85219, #55418, #49242, #15119, #7097, #80435, #42112, #43074, #6634, #43981, #8004, #63945, #6161, #14213, #14675, #93255, #71978, #51095, #86602, #79536, #92783, #29338, #72879, #78595, #35968, #35515, #87076, #43531, #71028, #49699, #27952, #72428, #29802, #35031, #21292, #13737, #50648, #42587, #79982, #7545, #58683, #36895, #64888, #21771, #452, #56842, #93713, #22225, #28868, #57756, #65812, #57300, #36429, #65345, #58232, #64429, #922, #87527, #85683, #22674, #51546, #20830, #71502, #28409, #86142, #50165, #79062, #66707, #9387, #30723, #73810, #45840, #2771, #25020, #10323, #88923, #39190, #16054, #15580, #16510, #68102, #61014, #44907, #89860, #9865, #17454, #1836, #8469, #59623, #67183, #3227, #32118, #52947, #88471, #24071, #37349, #73357, #66256, #53892, #1371, #30253, #44450, #31653, #31199, #45361, #60543, #24536, #59144, #89381, #87988, #81824, #52023, #23141, #37801, #80909, #16975, #53420, #8923, #23618, #52485, #74744, #82303, #38740, #67645, #46304, #38271, #81360, #74264, #2318, #75208, #60084, #83690, #82760, #61934, #4630, #54812, #18851, #62893, #91252, #83223, #55306, #25470, #5584, #90770, #12201, #69499, #55769, #69042, #32594, #41531, #84159, #17912, #47709, #77541, #18368, #3709, #46763, #47228, #76608, #91729, #92194, #11732, #26416, #33503, #77070, #63364, #48639, #40585, #62410, #12691, #70457, #19307, #48169, #76138, #84622, #26882, #25929, #19770, #41044, #39649, #75664, #69972, #5112, #34455, #33990, #27350, #10788, #68572, #61484, #90316, #54349, #11272, #40125, #4171, #33044, #86958, #21644, #43412, #79420, #49585, #58113, #85568, #57182, #78021, #27833, #6514, #50522, #20249, #56722, #22111, #72307, #43864, #20715, #78481, #35392, #72761, #14087, #13617, #64312, #14555, #7428, #6044, #56236, #36308, #42470, #93137, #71380, #50980, #28292, #28752, #93594, #65224, #86023, #21172, #79865, #49125, #50041, #13161, #328, #29214, #41997, #6979, #15005, #78936, #807, #85099, #42952, #71858, #7882, #36773, #70911, #34916, #35852, #57635, #64769, #86478, #65693, #63828, #92661, #80321, #16855, #60426, #66142, #88352, #87871, #74623, #31080, #58571, #37238, #51432, #2196, #17338, #67985, #8806, #1258, #38143, #30140, #67529, #59968, #46189, #2659, #1714, #9266, #81706, #87411, #23503, #9752, #59500, #81246, #24416, #44794, #88806, #30598, #52371, #23020, #31538, #23953, #22558, #38626, #67060, #16393, #52828, #75094, #51899, #45244, #37687, #80792, #74149, #73697, #15940, #45710, #89266, #39072, #53296, #82182, #10203, #59024, #29687, #15460, #44333, #73244, #66593, #8355, #91125, #4988, #83103, #89737, #18256, #54694, #32475, #76495, #33874, #62783, #76958, #90205, #48053, #12086, #84509, #25814, #32929, #41415, #83568, #18730, #3111, #61372, #4513, #3585, #76016, #68450, #91616, #25354, #69381, #40463, #26296, #47109, #54234, #26771, #60886, #11149, #53779, #55190, #62289, #24899, #47591, #69854, #61821, #31994, #82646, #4059, #40011, #55656, #19655, #17795, #46648, #68928, #33390, #90653, #11618, #40934, #84048, #19194, #75550, #48524, #77425, #39529, #12564, #10674, #21530, #71752, #5474, #77912, #92082, #42835, #57999, #14905, #49482, #13054, #78831, #41890, #14455, #6878, #86855, #43312, #42360, #49935, #28645, #34344, #35272, #50410, #6400, #28188, #65122, #85465, #35751, #71273, #64201, #34808, #72208, #64664, #63251, #79316, #13977, #93032, #93492, #22011, #63721, #57077, #78372, #27714, #85916, #20612, #92546, #57535, #86379, #79763, #225, #7325, #29105, #70801, #70348, #21067, #50881, #27237, #5936, #56125, #36203, #84978, #56613, #20129, #13511, #49014, #73128, #23401, #74507, #9638, #23854, #37136, #88706, #52720, #32713, #66494, #73594, #83340, #1611, #59390, #43761, #8255, #45144, #51790, #66948, #2087, #87309, #72660, #30977, #16750, #81602, #22920, #38525, #88242, #702, #7781, #52267, #37583, #68701, #81147, #59865, #65587, #16291, #3831, #36667, #80680, #61598, #29586, #44220, #58465, #90431, #9161, #45605, #25587, #66044, #54470, #1156, #44693, #22456, #15360, #87768, #38040, #51329, #30039, #80222, #58920, #15836, #8705, #30496, #74043, #35045, #70109, #83822, #42125, #71042, #55895, #91385, #27007, #40245, #76266, #69161, #56856, #4288, #11393, #18486, #5707, #34119, #48295, #34583, #27478, #33166, #63492, #27967, #91853, #54942, #63959, #40705, #62057, #19896, #92323, #90892, #47349, #26055, #84749, #56370, #48767, #77673, #12826, #12326, #92799, #18974, #47827, #41665, #76729, #19432, #11856, #26541, #63021, #84281, #77197, #85234, #70582, #69625, #20385, #4753 ),
 ( #49255, #33633, #55428, #62543, #78150, #41170, #13288, #5249, #6176, #65360, #80449, #86157, #85697, #86618, #44467, #37363, #21308, #66270, #79997, #87541, #71994, #78609, #7112, #43545, #50181, #467, #22688, #51561, #65830, #79077, #36912, #937, #73372, #14690, #21788, #30267, #72442, #7560, #20843, #14229, #87091, #4, #15134, #43997, #35531, #49714, #72894, #43090, #64903, #57315, #15594, #35983, #58248, #29356, #8018, #28884, #57772, #8484, #13754, #50664, #42602, #29816, #51111, #71517, #36445, #58697, #79550, #6651, #64444, #22240, #1385, #93270, #28424, #80926, #23156, #31214, #31667, #16525, #88938, #68117, #9880, #2786, #16069, #46320, #89875, #1851, #24087, #23634, #10338, #60560, #88003, #66723, #44923, #89398, #46778, #3724, #38286, #30738, #67660, #59640, #3243, #24552, #75679, #32133, #60099, #38756, #17470, #52040, #52963, #39205, #81840, #16990, #53907, #74279, #53436, #45855, #74761, #52499, #61029, #82320, #73825, #25036, #75224, #82775, #17927, #10804, #81376, #39666, #67199, #45376, #68588, #9402, #2335, #59159, #8938, #37816, #88487, #84174, #4186, #56254, #85114, #69988, #11747, #41062, #54364, #90331, #83238, #70928, #18385, #25485, #32610, #19786, #48184, #62426, #48657, #41547, #47242, #77558, #42012, #12216, #69057, #78037, #54827, #76154, #34005, #12707, #11287, #61499, #40141, #5128, #70471, #62909, #91745, #26896, #26431, #49140, #33060, #61949, #55784, #90786, #33520, #25946, #40600, #77085, #4645, #91267, #5599, #84637, #83705, #34473, #18867, #13177, #69514, #63379, #19322, #92209, #47724, #76624, #20264, #27365, #55324, #64784, #821, #6531, #20730, #63846, #35407, #6995, #15019, #15477, #71873, #43427, #21661, #345, #80335, #65709, #35867, #50537, #29702, #58585, #93609, #79435, #64327, #72775, #43879, #78954, #36789, #14571, #56737, #92678, #72322, #28767, #87424, #7443, #58127, #27848, #36325, #22572, #85583, #14104, #51446, #49600, #93153, #6059, #44348, #65239, #86972, #29232, #28308, #7900, #57197, #57650, #78496, #71398, #50058, #22126, #13634, #86038, #34931, #50994, #42485, #21187, #42968, #86498, #79879, #53313, #59983, #8370, #81262, #89280, #80805, #30153, #37251, #15953, #23516, #38641, #75108, #52385, #31095, #38162, #52844, #10218, #24431, #16407, #67077, #60444, #82198, #45259, #2211, #44809, #2673, #67544, #59517, #31552, #88822, #1271, #66155, #23970, #74163, #17352, #81721, #16870, #59036, #45729, #46203, #87883, #88366, #73258, #73710, #30615, #23036, #51914, #8820, #37700, #66606, #74639, #1728, #9766, #9279, #85886, #35720, #14422, #29552, #28159, #64634, #30004, #51297, #51757, #28615, #93462, #43279, #80646, #21977, #57504, #87735, #22887, #7749, #72177, #72629, #21038, #57050, #49906, #8670, #78801, #13946, #64169, #80189, #79733, #192, #15329, #73094, #42803, #44189, #73561, #43729, #6846, #15801, #86348, #71719, #65554, #8224, #21499, #93001, #50377, #36633, #37102, #668, #58432, #87278, #57965, #44660, #79281, #7293, #22425, #36173, #65092, #29073, #86819, #14875, #50850, #66011, #1123, #58889, #38002, #10070, #74008, #54091, #45566, #60747, #24277, #10529, #81113, #90066, #38938, #66459, #2522, #32329, #66912, #52230, #1577, #2050, #38488, #46512, #46968, #9601, #74958, #53152, #31858, #18116, #3434, #67394, #82033, #61231, #25218, #31399, #17191, #30941, #39396, #75413, #16711, #68311, #46053, #88206, #30459, #67847, #60289, #82963, #2973, #89588, #59354, #24759, #75870, #23363, #74470, #37548, #16256, #59829, #45106, #9125, #53641, #82511, #17659, #88670, #23819, #52682, #89126, #81563, #76351, #55037, #70199, #68785, #11477, #70658, #91933, #92400, #69243, #40327, #83905, #27560, #62632, #4371, #34661, #63575, #48379, #19057, #19511, #32791, #3914, #61679, #49334, #90511, #25674, #10994, #27087, #26623, #40790, #55974, #19977, #54553, #84828, #20467, #84362, #47442, #56455, #33249, #83421, #12411, #48853, #18576, #39863, #62146, #77281, #77759, #41261, #5332, #34200, #4838, #85317, #90975, #26141, #63105, #47912, #11941, #76815, #69707, #55513, #33721, #91472, #12907, #41745, #5787, #50739, #20921, #1015, #86232, #7635, #64978, #51186, #64521, #22771, #78228, #79160, #42679, #80073, #44072, #6252, #42208, #50253, #79623, #35606, #14307, #87166, #28960, #21864, #35120, #65435, #15216, #49790, #43168, #71597, #29432, #14765, #13367, #85771, #64041, #43618, #65902, #71122, #57390, #78687, #86700, #13828, #22315, #72515, #29894, #72974, #72069, #57846, #36519, #92883, #7186, #58323, #36061, #81, #8103, #93347, #549, #36990, #58778, #6732, #87620, #28044, #56934, #28498, #21384, #81454, #74845, #3321, #16145, #16603, #30823, #9015, #45458, #66799, #44997, #81918, #38830, #61117, #46400, #31291, #75300, #52120, #51641, #52574, #10419, #32211, #81002, #89956, #45937, #53524, #37894, #44546, #1929, #9481, #73899, #60177, #82400, #17548, #31746, #59720, #2863, #60639, #39283, #74358, #38367, #80527, #67281, #2411, #15680, #88563, #53043, #23711, #9958, #67737, #1462, #73449, #89477, #89015, #24162, #23240, #68201, #17070, #24637, #8559, #37439, #66348, #30348, #59238, #88084, #40219, #75762, #48269, #84256, #82854, #69597, #91826, #83791, #34093, #4263, #55870, #4727, #10883, #18006, #33605, #18946, #84722, #40679, #77171, #46859, #62513, #19871, #39746, #33141, #48741, #68671, #25563, #25111, #77645, #19406, #12301, #41145, #18461, #26980, #54443, #26029, #3806, #90406, #69135, #70078, #32687, #83316, #12796, #5220, #41637, #47320, #76236, #62031, #70556, #76702, #11368, #5679, #34554, #91353, #90865, #26514, #61573, #54912, #47801, #63463, #11828, #55403, #53985, #62995, #14198, #28393, #79522, #7530, #85203, #14661, #7988, #71963, #35015, #43964, #20815, #13260, #93699, #43516, #56341, #27449, #42097, #64873, #72414, #28855, #7081, #57741, #86127, #15104, #92768, #27935, #35954, #78122, #93240, #92292, #71486, #43059, #64413, #57285, #36415, #86586, #56826, #21757, #63930, #72863, #6618, #50632, #79047, #65331, #78580, #71012, #51079, #435, #20353, #21276, #87060, #85667, #6144, #49225, #49685, #50148, #29323, #36882, #58216, #22209, #79967, #13718, #42571, #35498, #15996, #30659, #45774, #9808, #80848, #59561, #44391, #52886, #22612, #31597, #8411, #862, #81304, #67122, #43920, #15058, #29743, #52429, #2257, #16450, #88410, #45302, #73751, #2717, #80375, #15516, #23561, #65753, #44848, #79921, #59084, #1775, #51957, #8863, #60027, #74207, #73299, #9325, #51487, #60486, #87926, #38208, #66649, #81766, #66196, #58624, #38682, #31140, #72815, #37741, #74685, #37289, #87465, #7941, #1312, #88864, #24013, #89323, #16916, #67587, #24478, #36835, #30194, #23077, #83162, #4116, #20552, #78312, #54291, #32988, #17855, #27650, #63660, #32538, #85404, #61879, #10263, #17398, #90710, #47170, #49422, #68986, #12992, #75151, #27175, #13451, #46247, #61431, #42302, #39133, #53838, #53357, #71211, #20065, #41830, #77844, #46706, #56549, #82704, #18314, #68044, #24962, #3648, #48946, #3171, #75609, #6338, #70741, #35209, #10733, #39589, #90263, #64137, #11211, #68512, #92970, #82243, #56062, #25412, #84915, #32055, #60949, #89800, #76079, #40068, #5875, #34745, #92483, #57930, #7263, #65517 ),
 ( #65979, #7716, #51264, #21467, #85853, #50343, #160, #93430, #21945, #80157, #15295, #58400, #28582, #29520, #636, #8189, #29039, #36140, #29971, #86786, #50818, #28128, #57474, #43697, #43249, #36600, #87246, #42767, #57017, #22392, #86315, #72147, #79249, #73059, #14390, #72596, #44152, #37070, #65059, #79702, #1090, #49873, #14844, #71686, #21006, #78771, #6816, #13912, #35690, #64604, #57317, #18977, #19898, #77198, #20845, #78610, #40707, #76731, #84750, #85238, #70113, #48769, #27968, #63493, #56371, #69627, #6178, #49716, #55431, #77676, #12328, #63961, #20386, #47829, #26542, #4755, #49258, #6654, #11858, #91855, #84283, #27480, #19433, #56858, #78152, #35532, #85700, #12829, #92324, #71044, #33635, #41666, #92802, #70584, #5710, #13756, #34120, #13290, #34586, #42127, #41172, #42604, #35046, #62545, #71519, #64446, #93272, #28425, #91388, #48297, #5251, #63023, #27009, #55896, #86158, #65362, #8022, #58250, #87094, #66274, #941, #86620, #58701, #28885, #8942, #469, #15598, #72897, #59162, #72443, #35984, #44927, #87544, #21309, #51114, #80929, #21790, #7115, #50182, #50665, #22244, #1388, #1854, #80000, #29819, #36917, #80452, #66727, #52045, #15138, #65833, #16073, #73829, #44000, #22691, #79551, #88008, #30271, #29359, #23161, #51566, #43091, #79079, #44471, #73375, #37820, #8487, #37366, #14232, #30743, #71996, #64904, #5, #57773, #14692, #43547, #7561, #36447, #25039, #46782, #82779, #52967, #61503, #88942, #60564, #81380, #31218, #9885, #53911, #23638, #60103, #25490, #75683, #47246, #24090, #81844, #38760, #76159, #17474, #16994, #83242, #18389, #3246, #67664, #68121, #16528, #52503, #45380, #4190, #9406, #38291, #59646, #10808, #75228, #89402, #68593, #3729, #67206, #32613, #69061, #39208, #2339, #11292, #45860, #74767, #61034, #90335, #2790, #88491, #31671, #32137, #54368, #17931, #40145, #24556, #53441, #82324, #46325, #10342, #49605, #41067, #56260, #19792, #6064, #19326, #76628, #85588, #5604, #61954, #91749, #27853, #33524, #47728, #90790, #62430, #34011, #42017, #42490, #5132, #70476, #48661, #27370, #13639, #92684, #62913, #77563, #56744, #20735, #26900, #12711, #91271, #34936, #70933, #12220, #63851, #41553, #83710, #25950, #34478, #55788, #78501, #63384, #85119, #54831, #92214, #71403, #18872, #69992, #33065, #11751, #26436, #40604, #69518, #20270, #49146, #78042, #55328, #4650, #84178, #84641, #48188, #77090, #13183, #65715, #64333, #7000, #66161, #87431, #87890, #64789, #35873, #50542, #23042, #58132, #71879, #30160, #59042, #43884, #79440, #15025, #28313, #93159, #57202, #44814, #86043, #21192, #6536, #22577, #22131, #36330, #51452, #15483, #50063, #80341, #15959, #79884, #42973, #51920, #28772, #78959, #7905, #44354, #14109, #35413, #93614, #72780, #73264, #36795, #827, #29708, #350, #80810, #57655, #86503, #58591, #21666, #7448, #14577, #43432, #51000, #72328, #65244, #8376, #37256, #29237, #86977, #1277, #16413, #25373, #2217, #88372, #75114, #60911, #37706, #8826, #23522, #46210, #89758, #10224, #53319, #39091, #67550, #90223, #74169, #9286, #82204, #59523, #74645, #73716, #52850, #89285, #45735, #9772, #53796, #17358, #38168, #68004, #45265, #54253, #81727, #3133, #60450, #46666, #59988, #52391, #32494, #32013, #66612, #38647, #68472, #67084, #81268, #1734, #31101, #2679, #82665, #83123, #31558, #24920, #24437, #17813, #18274, #39549, #75570, #10692, #3607, #61392, #30622, #88827, #23976, #16876, #56143, #26315, #77928, #91635, #4078, #11170, #26789, #40951, #13071, #62800, #5491, #68947, #55675, #41907, #40030, #55210, #70820, #32948, #47611, #47128, #5952, #12588, #34364, #70366, #40484, #49032, #76514, #48072, #61841, #18753, #91149, #41434, #90673, #11637, #34824, #63269, #63737, #69400, #4533, #84064, #92563, #5011, #33409, #27734, #56631, #84526, #19213, #19674, #25833, #54712, #83590, #85481, #62308, #76976, #76041, #92100, #48542, #12105, #27256, #84995, #69872, #20151, #33893, #77443, #42377, #78388, #71289, #58935, #6416, #13528, #20628, #7796, #36219, #50430, #36681, #29602, #35292, #65604, #30054, #240, #57093, #66059, #42855, #64218, #22027, #717, #93049, #49498, #28205, #86872, #58481, #50896, #29121, #79779, #14470, #37152, #21083, #49954, #58018, #85933, #21546, #78846, #93506, #65139, #86394, #79335, #87325, #14922, #13992, #43775, #71770, #1172, #28662, #72677, #7339, #22473, #6892, #35767, #73148, #51346, #64680, #43327, #15375, #57549, #72225, #80238, #44237, #8272, #3025, #3493, #59883, #31453, #9660, #82087, #68364, #82564, #23871, #38544, #17712, #46565, #88723, #67447, #52284, #60803, #31911, #66966, #24813, #2575, #44710, #51807, #60342, #81619, #75464, #89179, #46106, #15852, #24331, #10585, #80701, #2106, #39448, #73611, #88262, #87786, #32386, #53208, #75011, #17246, #81164, #89642, #23419, #52737, #8721, #59407, #38057, #10123, #37599, #16308, #22936, #38989, #66509, #45160, #74059, #30996, #1629, #45622, #9179, #30511, #16768, #67902, #74525, #33303, #4896, #76871, #55572, #41804, #27146, #91031, #11997, #56032, #84886, #62201, #40846, #25724, #34256, #70257, #40379, #91993, #69765, #18170, #25272, #33781, #55096, #20037, #62696, #19568, #83018, #91526, #48915, #54149, #69296, #77816, #47023, #61734, #61286, #12965, #26682, #48434, #84420, #54608, #63162, #90566, #26201, #75926, #32844, #11532, #77338, #11052, #83479, #70715, #12472, #5846, #18636, #47503, #4425, #90120, #19112, #76410, #39923, #68842, #41320, #83963, #5391, #3970, #47967, #56518, #73029, #85377, #27620, #34718, #21917, #50314, #64578, #50791, #43672, #20526, #79675, #44125, #14362, #71182, #80126, #56989, #49395, #36114, #14817, #92457, #63632, #78286, #7238, #72567, #65031, #43221, #131, #28555, #51238, #35179, #64102, #72122, #13424, #35663, #42269, #13885, #79219, #6787, #93403, #7689, #29014, #92942, #57899, #6311, #15265, #42739, #86755, #21440, #36574, #20978, #28102, #87217, #65489, #85827, #57446, #29491, #49845, #78741, #71654, #86287, #606, #58374, #22364, #81052, #15735, #16651, #44597, #45991, #74407, #24693, #74896, #73948, #81504, #60226, #37040, #66850, #53090, #37941, #59770, #2911, #23296, #38422, #9063, #1985, #66398, #10007, #9537, #65954, #81969, #45505, #30876, #31339, #53576, #1514, #88611, #16195, #59292, #23758, #52170, #30400, #67331, #89065, #17599, #31795, #2463, #60689, #8612, #8157, #52622, #89529, #82451, #37488, #46449, #24215, #38878, #88138, #1065, #45047, #17125, #67785, #29944, #58829, #87674, #22825, #51693, #80582, #73500, #63045, #4313, #11416, #19920, #33191, #90914, #75351, #39801, #76753, #83362, #4777, #33659, #25159, #10466, #62568, #75809, #54494, #46908, #41199, #10933, #47851, #18998, #69649, #25611, #68723, #5273, #39332, #90454, #32262, #91409, #40732, #68250, #26080, #48321, #40267, #3374, #61168, #76290, #3853, #77222, #70137, #90004, #54033, #47376, #11881, #32733, #69184, #84304, #54969, #26564, #82900, #55453, #12350, #18056, #62081, #61622, #19454, #34142, #18512, #83845, #91876, #27030, #55919, #84771, #49278, #21331, #85260, #66627, #56880, #72019, #35554, #23057, #35066, #92345, #8843, #50201, #77700, #13776, #44828, #78173, #63517, #12849, #13311, #49737 ),
 ( #41687, #93294, #51935, #42625, #88388, #48792, #78634, #42149, #80825, #15976, #70605, #5732, #20866, #79105, #6199, #71544, #59058, #28445, #86180, #34607, #36007, #73731, #20408, #6677, #71067, #1292, #14254, #27500, #56398, #63986, #43112, #37721, #92826, #27989, #85721, #57338, #64467, #87906, #7136, #1752, #30639, #64925, #30174, #59538, #52409, #82221, #68488, #53335, #75131, #18290, #38662, #53815, #24457, #89301, #81744, #25389, #89775, #81284, #3624, #60928, #17375, #46685, #68963, #16895, #46227, #2695, #74663, #10241, #67566, #45752, #82683, #10710, #32964, #47148, #3150, #76056, #23993, #23539, #39110, #11186, #4093, #52866, #68023, #9787, #32512, #24938, #16430, #31118, #45282, #17833, #40046, #61857, #31577, #60004, #32033, #88844, #61408, #75587, #74185, #90240, #39567, #54269, #83139, #9304, #38185, #67100, #2234, #60466, #85496, #12122, #27271, #91652, #62818, #55227, #92582, #63284, #25848, #70835, #34379, #26805, #20166, #42392, #84082, #55691, #69890, #48089, #84542, #40967, #19231, #56158, #77942, #6434, #20643, #70381, #49513, #91167, #90688, #19689, #78405, #71304, #26334, #35308, #85015, #27750, #76993, #83607, #5028, #48558, #33909, #5509, #56646, #13544, #5967, #77461, #41924, #34841, #54730, #12603, #41449, #18769, #92117, #49047, #47627, #13086, #63752, #76531, #11653, #40500, #69419, #4550, #33424, #62328, #43341, #35780, #30067, #93519, #36699, #7809, #58494, #14483, #57564, #87800, #28220, #79348, #21100, #87339, #29616, #57108, #14935, #37165, #29138, #8737, #64234, #65152, #28678, #66074, #58952, #85948, #49968, #36234, #65619, #21562, #255, #73165, #43790, #730, #78859, #51361, #1186, #6905, #22949, #50445, #14010, #51823, #22488, #93064, #58032, #80715, #64693, #42869, #71783, #86407, #86886, #8285, #73625, #22040, #80252, #79793, #15388, #44725, #15869, #50909, #72690, #72238, #7352, #44254, #82104, #2120, #10603, #46580, #16782, #68379, #17262, #88276, #1644, #46121, #31469, #3510, #53222, #89659, #59425, #75024, #32401, #30524, #45636, #61300, #23432, #38072, #37614, #90136, #3041, #24827, #60816, #31010, #39462, #66983, #38558, #52300, #9194, #81635, #31924, #81177, #59897, #25286, #53711, #54163, #88739, #23885, #74545, #83032, #89194, #52753, #18186, #47038, #10137, #9675, #39003, #16321, #45173, #74075, #75939, #67460, #2589, #66525, #82578, #67917, #60357, #17725, #75478, #24347, #27159, #20538, #84433, #47517, #56533, #33318, #25739, #12485, #92006, #68854, #39937, #54621, #77351, #56047, #41336, #19581, #70270, #4909, #27634, #11545, #40392, #48450, #90579, #12011, #11068, #83977, #26696, #76884, #40861, #84901, #5404, #69310, #34269, #76423, #85389, #19125, #63176, #91540, #47980, #20050, #48931, #83493, #3983, #77828, #4438, #69779, #62214, #70727, #91044, #12978, #41816, #5859, #55111, #26217, #34730, #32858, #33795, #61747, #63646, #92468, #18651, #55585, #49408, #62709, #22838, #78298, #79232, #42751, #80139, #44136, #6323, #42284, #50325, #50801, #35675, #14373, #87228, #29024, #21928, #35191, #65499, #15279, #20990, #43234, #71668, #29503, #79686, #13437, #85839, #64118, #14828, #65965, #71196, #57457, #49857, #86767, #78756, #22376, #43682, #1076, #51249, #72132, #57911, #36585, #92954, #7248, #58385, #36124, #65041, #73041, #93415, #72578, #144, #7700, #6801, #8171, #618, #28114, #37054, #29956, #58841, #87685, #57002, #64590, #13897, #86300, #28566, #21452, #66861, #16209, #81980, #38889, #61179, #46461, #31351, #75363, #52182, #51705, #52635, #10478, #3385, #81064, #32273, #46003, #53590, #37954, #44609, #1996, #9548, #45060, #60239, #82462, #17610, #31808, #73960, #2923, #60701, #39344, #74419, #81515, #90016, #38435, #67343, #80593, #9074, #53103, #23770, #89541, #89077, #30889, #24226, #88151, #68263, #59781, #74907, #2474, #24704, #88623, #1526, #15750, #17137, #73514, #16662, #8623, #45517, #66409, #37500, #10019, #67798, #30412, #59303, #23310, #62580, #40743, #19465, #5743, #84783, #54982, #69660, #19933, #48801, #26093, #4791, #83378, #91886, #34153, #4326, #55929, #33670, #75823, #82914, #91422, #19010, #77710, #26575, #77233, #46921, #55464, #12860, #18068, #33203, #41698, #10947, #25624, #25170, #70616, #84314, #12363, #48332, #18526, #27040, #54506, #83858, #39813, #90467, #69197, #41210, #68735, #47392, #34618, #70148, #63528, #76303, #11428, #62094, #54044, #76766, #40280, #3866, #32746, #5284, #90928, #63057, #61634, #47863, #11894, #36950, #49287, #85270, #92355, #79583, #14265, #28456, #14725, #7592, #20419, #43578, #8058, #72029, #35079, #44031, #20877, #13321, #38, #72476, #56409, #27516, #42161, #64937, #36478, #28918, #7145, #57806, #86191, #15173, #92836, #27999, #36019, #78183, #93306, #71078, #71554, #43125, #64478, #86656, #49749, #57351, #65395, #21821, #50696, #6210, #507, #29390, #63997, #21343, #56891, #58282, #87124, #85731, #78646, #13786, #22276, #80032, #42638, #6690, #35565, #51148, #50214, #72933, #79117, #82357, #9919, #37856, #45417, #24124, #971, #30781, #17032, #1890, #23671, #60599, #80962, #2372, #66760, #59680, #30307, #67696, #38328, #29852, #45897, #9442, #88523, #88976, #17505, #59195, #52537, #44958, #23198, #81412, #16106, #88043, #31250, #53003, #75259, #89434, #74317, #24592, #66308, #65863, #16562, #53480, #46358, #1423, #10374, #60137, #2824, #52079, #58736, #73858, #67242, #8976, #81877, #31707, #87579, #74802, #38792, #22723, #51598, #80486, #15634, #44503, #73409, #8519, #37398, #39241, #3760, #40632, #47277, #62464, #91305, #82810, #68157, #26468, #39703, #18417, #10839, #5168, #68626, #11782, #76655, #33554, #83273, #32645, #62946, #3277, #54400, #89913, #55357, #4680, #32170, #83745, #12251, #4219, #77596, #61070, #40174, #61533, #41097, #34043, #25069, #53941, #11323, #70026, #17961, #76193, #91780, #46814, #90364, #75716, #26931, #84209, #19356, #48220, #25521, #55819, #69093, #33094, #61985, #90820, #25980, #77122, #54865, #18902, #84675, #19824, #48690, #47757, #69550, #56780, #29274, #64369, #78073, #36367, #65280, #50099, #85622, #21230, #34511, #70509, #63418, #51033, #92247, #5636, #12745, #93649, #28347, #42524, #28809, #21705, #27404, #57693, #22165, #86079, #49179, #58169, #34970, #56292, #14148, #86536, #85156, #41587, #20308, #78993, #50581, #43012, #71916, #7037, #6573, #87013, #13216, #42052, #35907, #70966, #13674, #6098, #20768, #57237, #78535, #71436, #79476, #64825, #63884, #14611, #92720, #27890, #49640, #43468, #93195, #72365, #35450, #7482, #385, #82896, #45501, #75347, #11412, #17121, #31335, #74403, #45987, #17595, #25607, #26076, #82447, #54029, #32258, #10929, #90910, #76286, #46445, #61163, #40263, #69180, #10462, #90000, #74892, #83358, #54490, #89525, #47372, #25155, #67327, #9533, #18052, #39328, #4309, #46904, #68719, #38418, #75805, #68246, #39797, #67781, #3370, #18508, #3849, #32730, #2459, #61618, #33187, #53086, #90450, #10003, #62077, #54965, #60222, #24211, #89061, #16647, #81965, #38874, #53572, #2907, #31791, #60685, #27984, #56393, #6672, #56875, #55914, #63512, #42144, #18994, #48787, #35061, #19916, #41682, #78629, #5268, #20403, #84766, #77695, #48316, #85716, #85255, #47847, #63981, #27495 ),
 ( #49273, #26560, #35549, #91871, #13306, #70600, #20861, #70132, #33655, #42620, #78168, #76749, #12844, #13771, #84300, #4773, #11877, #19450, #5727, #92821, #93289, #34602, #71062, #92340, #6194, #64462, #49732, #71539, #28440, #83841, #40728, #69645, #62564, #77217, #91405, #55449, #63040, #12345, #41194, #34137, #27025, #8040, #51134, #23179, #956, #37381, #79100, #29835, #52062, #21326, #65378, #80944, #43107, #57790, #57333, #16089, #50196, #59178, #66742, #58718, #23, #8957, #79567, #72014, #87562, #44941, #14249, #86175, #7131, #37836, #1868, #36002, #64920, #28902, #80017, #86640, #21808, #50681, #14710, #43563, #58268, #72459, #36463, #7578, #44016, #490, #10823, #39221, #31232, #3260, #67223, #47260, #38774, #53925, #17487, #3744, #17008, #74297, #83257, #32150, #59662, #89416, #25503, #60118, #45398, #88505, #88957, #31686, #39683, #40158, #2804, #68139, #46339, #25052, #11306, #90347, #60581, #75241, #54381, #18401, #24570, #10356, #24104, #32626, #68607, #9900, #61516, #61051, #81394, #23652, #89894, #53458, #76174, #82793, #17945, #52518, #46796, #69075, #16542, #67678, #30760, #9421, #52985, #38308, #2354, #75698, #81859, #45877, #74783, #82339, #33538, #5149, #25963, #69532, #48202, #63401, #61967, #4665, #63867, #85135, #85605, #62443, #91286, #77104, #20752, #55803, #26452, #27871, #56764, #41570, #12235, #12727, #54844, #90804, #83726, #42508, #18886, #47741, #4203, #20290, #19807, #34026, #49164, #13199, #76639, #77576, #34955, #11764, #41082, #92701, #40616, #55341, #33078, #49623, #92230, #78057, #27386, #84192, #6081, #19340, #62930, #70006, #91764, #26916, #56276, #84655, #48675, #78519, #42035, #13656, #70492, #5620, #34495, #70949, #29253, #42993, #2587, #31467, #15040, #50561, #79902, #93179, #35431, #28331, #17260, #57221, #64353, #71420, #59895, #86995, #7464, #88737, #81633, #86061, #23883, #82101, #51015, #14128, #24345, #93632, #21211, #72797, #52751, #50081, #6552, #78976, #43900, #16780, #7921, #36812, #65733, #65261, #89192, #71899, #7019, #844, #35890, #72346, #64808, #79458, #22147, #43449, #36347, #45634, #29725, #28789, #74542, #57676, #53220, #14592, #9673, #58149, #38556, #86519, #21684, #60355, #67458, #367, #3039, #53709, #10135, #75022, #46119, #31922, #60814, #39001, #67915, #89656, #24825, #82576, #35870, #22129, #7446, #71401, #86041, #36328, #65242, #42488, #21190, #6062, #14574, #50540, #20733, #72325, #50061, #92212, #5602, #78957, #35410, #348, #57200, #93612, #14107, #34934, #43430, #79438, #49603, #29235, #42971, #27368, #34476, #71876, #64330, #58130, #6998, #28770, #63382, #64787, #86975, #56257, #78499, #50997, #85117, #42015, #41550, #79882, #57653, #86501, #21664, #63849, #70474, #70931, #6534, #20267, #13180, #85586, #49143, #78040, #92681, #27851, #56740, #13637, #93156, #28311, #59040, #31556, #66609, #80339, #38645, #67548, #52389, #87887, #23520, #36793, #72778, #65713, #53317, #825, #7903, #15022, #2215, #30619, #44812, #31099, #23974, #29706, #59986, #24435, #88370, #51449, #60448, #37254, #58589, #16411, #88825, #87428, #43882, #22575, #81266, #52848, #45263, #74167, #9283, #8824, #89283, #15481, #44352, #38166, #73262, #15957, #8374, #23040, #59521, #80808, #73714, #81725, #67081, #66159, #16874, #1275, #30157, #51918, #45732, #1732, #74643, #37704, #9769, #2677, #54710, #17356, #47126, #76973, #82662, #3131, #46207, #17811, #83121, #91146, #91633, #54251, #25831, #4075, #76512, #62798, #48070, #18272, #32946, #12103, #40948, #76039, #61838, #69870, #5008, #11168, #90671, #46664, #55208, #26313, #61389, #19211, #83587, #39089, #75112, #18751, #40028, #33891, #47609, #40481, #10222, #11635, #26787, #68002, #90221, #82201, #32011, #75568, #60909, #89756, #69398, #4530, #33407, #10690, #84062, #39547, #68945, #24917, #53794, #32492, #62306, #68470, #3605, #25370, #42852, #72222, #13069, #84993, #92561, #48540, #42375, #27254, #79332, #12585, #93046, #85479, #64216, #41432, #70364, #5489, #34362, #63267, #92098, #56140, #71768, #71287, #20626, #64678, #28660, #41905, #21544, #70818, #35289, #49497, #78386, #6414, #28203, #57091, #50427, #85931, #21081, #49952, #1626, #16305, #59404, #37596, #23416, #22934, #45619, #29600, #58479, #81161, #14919, #87784, #29119, #8270, #44707, #1170, #51804, #9176, #38054, #87323, #66963, #715, #74521, #37150, #30993, #73608, #59880, #15373, #72675, #38541, #88720, #58015, #80696, #23868, #22471, #51343, #22025, #44235, #52734, #67444, #79776, #73144, #66057, #18167, #90563, #76868, #62198, #32382, #82083, #3022, #2571, #33300, #61731, #83476, #25721, #89638, #4422, #31908, #3489, #24328, #67899, #46562, #54605, #60339, #60800, #91028, #18632, #83960, #24808, #53694, #75461, #19109, #54146, #82561, #26197, #55091, #39918, #10582, #11048, #53205, #89176, #17241, #40842, #46103, #75008, #31450, #47498, #47020, #61283, #76407, #11529, #10120, #40376, #11993, #75922, #38986, #47964, #17709, #39445, #3967, #69293, #68361, #90117, #25269, #68839, #83015, #32841, #49390, #35175, #63628, #86283, #70252, #5387, #78282, #55568, #70711, #69761, #48910, #85372, #41800, #5842, #49841, #13420, #34252, #42265, #12468, #21436, #77812, #92937, #56513, #42734, #56027, #19564, #28551, #71178, #4892, #34714, #64574, #63158, #84416, #33776, #91989, #92453, #78738, #79215, #27616, #6307, #20522, #64097, #50310, #35659, #28098, #56985, #93399, #57442, #85823, #20974, #27142, #71649, #13881, #12961, #6782, #14358, #26678, #62689, #91522, #48430, #77334, #41315, #84882, #20033, #22820, #73944, #7235, #51235, #9059, #36110, #15262, #15731, #603, #73025, #52165, #87670, #80578, #128, #30396, #37937, #79673, #8153, #7686, #88134, #44592, #72119, #50788, #65028, #73496, #30872, #81500, #22361, #14814, #51689, #43669, #81048, #8608, #59766, #16191, #44121, #37484, #1510, #29011, #37036, #23292, #65950, #1061, #66846, #58371, #66394, #29940, #58825, #36571, #45043, #59288, #57896, #1981, #88607, #23755, #52618, #43218, #65486, #86752, #80123, #29486, #21914, #87213, #72564, #85732, #42639, #64938, #50215, #35080, #79118, #84784, #55466, #56410, #14266, #7146, #19934, #36021, #49750, #57352, #41700, #48333, #70617, #13322, #48803, #63998, #86192, #21344, #35566, #77711, #6691, #64480, #43126, #78184, #85271, #39, #42163, #71079, #84315, #12861, #56893, #63529, #78647, #13787, #5285, #19466, #71555, #5744, #34619, #27041, #72031, #92356, #28000, #92837, #93307, #27517, #20420, #77234, #12364, #49289, #41211, #28457, #20878, #70149, #6211, #34155, #63058, #91887, #28919, #29853, #87126, #30782, #88524, #50697, #45418, #29391, #58283, #37399, #14726, #58737, #57807, #8059, #44504, #972, #87580, #8977, #66309, #22277, #1424, #65396, #74318, #36951, #52080, #15635, #1891, #15174, #72477, #81413, #30308, #86657, #22724, #23672, #51149, #43579, #21822, #80033, #51599, #37857, #38329, #80487, #59196, #73410, #23199, #9443, #52538, #8520, #88044, #16563, #67243, #80963, #16107, #44032, #59681, #66761, #65864, #79585, #44959, #7593, #36479, #73859, #508, #72934, #17962, #54401, #24125, #75717, #33096, #60138, #10375, #61987, #81878, #2825, #2373, #90822, #61534, #83274, #25522, #89435 ),
 ( #53004, #40634, #17033, #88977, #31251, #18418, #46815, #32171, #47278, #11324, #45898, #76194, #11784, #10840, #38793, #47759, #24593, #74803, #3761, #40175, #9920, #67697, #31708, #68627, #69094, #32646, #39704, #90365, #89914, #25982, #60600, #53481, #3278, #54867, #76657, #82358, #17506, #4221, #83747, #46359, #75260, #39242, #53942, #68158, #18904, #61071, #25070, #82811, #62948, #20770, #49642, #57239, #92249, #5638, #14150, #27406, #85158, #69552, #34045, #70968, #77598, #92722, #27892, #19358, #4682, #56782, #70028, #48692, #41099, #35452, #5170, #42054, #13218, #63886, #19826, #91782, #93197, #33556, #84677, #26470, #85624, #34972, #62466, #20310, #42526, #34513, #91307, #55359, #70511, #26933, #71438, #64371, #84211, #48222, #41589, #6100, #55821, #63420, #78537, #49181, #13676, #77124, #6575, #28349, #12253, #56294, #12747, #86081, #21232, #78075, #50101, #78995, #16801, #31944, #82595, #22167, #50583, #52774, #79478, #82125, #45657, #60835, #17282, #16341, #23903, #2607, #71918, #9213, #89214, #74094, #2139, #39021, #58171, #74565, #45191, #38093, #7484, #46139, #9694, #7039, #24365, #81653, #67003, #67478, #89679, #36369, #31028, #51035, #387, #59915, #87015, #65282, #38575, #31487, #53729, #67936, #60375, #88757, #3059, #43470, #57695, #35909, #72367, #53243, #75042, #43014, #10154, #24846, #64827, #93651, #28811, #86538, #21707, #14613, #29276, #81195, #18669, #62230, #75957, #84448, #26712, #90596, #48466, #91061, #68397, #75495, #26235, #11560, #77366, #33333, #69794, #39477, #55128, #12502, #10619, #25756, #41354, #3527, #18202, #17742, #70286, #76899, #4927, #40876, #11088, #19598, #47054, #47535, #32417, #83050, #61763, #12029, #61316, #39954, #5419, #33813, #34284, #68870, #4000, #54637, #63192, #69326, #32875, #92022, #27177, #83993, #83511, #19140, #90154, #25302, #54180, #56064, #76439, #40408, #46596, #62725, #47995, #4455, #91555, #55600, #77846, #7265, #638, #64606, #27652, #36602, #13453, #5877, #86317, #72149, #48948, #20067, #34747, #57476, #36142, #21469, #93432, #50345, #78773, #7718, #85406, #20554, #28584, #70743, #85855, #84917, #64139, #6818, #57019, #21008, #65061, #79251, #49424, #14392, #56551, #65519, #92972, #43251, #71688, #57932, #71213, #63662, #43699, #162, #12994, #78314, #49875, #42304, #29041, #86788, #41832, #92485, #6340, #21947, #72598, #29522, #28130, #35211, #50820, #13914, #79704, #14846, #42769, #35692, #30427, #37969, #16678, #87248, #23328, #9565, #88169, #16224, #53118, #73529, #88638, #59318, #52198, #22854, #60255, #30907, #22394, #38453, #2014, #81080, #81530, #10034, #51720, #45075, #37515, #15768, #73975, #8638, #80610, #23786, #45533, #67813, #81998, #66877, #17154, #58857, #58402, #9092, #46020, #38904, #87703, #2938, #52650, #89092, #44627, #51266, #66425, #59797, #1544, #74434, #24244, #74923, #67359, #2489, #31366, #80159, #15297, #44154, #73061, #8191, #37072, #65981, #1092, #29973, #33215, #39826, #54999, #83871, #75379, #31824, #19023, #32290, #10959, #3399, #91437, #61195, #4338, #69209, #26106, #75836, #25184, #55479, #89554, #46934, #82477, #47877, #90942, #24722, #76316, #4805, #90479, #70163, #60715, #32758, #90032, #33685, #26589, #53606, #17624, #3880, #62111, #82927, #61646, #40756, #11442, #76780, #46475, #11907, #62594, #10492, #84328, #69674, #39361, #25636, #19478, #54057, #68277, #18080, #68750, #54520, #48345, #41224, #83389, #77248, #47406, #12377, #18539, #40293, #55940, #84796, #12873, #41712, #27054, #19946, #63070, #77723, #5298, #48817, #34168, #91900, #51363, #58496, #45175, #88279, #31471, #16324, #52755, #22490, #74077, #60359, #87341, #8739, #89196, #80254, #1188, #732, #24349, #59899, #81637, #23887, #87802, #2591, #30069, #1646, #15390, #66076, #44727, #88741, #44257, #58954, #53224, #16784, #82106, #22951, #51825, #73627, #17265, #52302, #80718, #46123, #75026, #38074, #37616, #9196, #73168, #8287, #37167, #39005, #15871, #66527, #29618, #45638, #66985, #30526, #74547, #9678, #59428, #38560, #10139, #2123, #23434, #81179, #31012, #67462, #69311, #55113, #31926, #3043, #82580, #40393, #83978, #4439, #47519, #33319, #61748, #84434, #68380, #3511, #76424, #53713, #68855, #67919, #47039, #83494, #39939, #3984, #47981, #11546, #32403, #62215, #10605, #19582, #75940, #91045, #54622, #40862, #54165, #26219, #89661, #19126, #4910, #60818, #11070, #33797, #17727, #61301, #24830, #62711, #76885, #12012, #69780, #90137, #91541, #25287, #32859, #46582, #39463, #18187, #26697, #75480, #83033, #55586, #48451, #77352, #90580, #25740, #18652, #12486, #92956, #12979, #65042, #145, #78757, #20539, #49858, #63177, #5405, #92008, #79687, #27160, #34270, #41337, #28568, #57003, #71197, #57458, #50326, #56048, #86301, #50802, #20992, #77830, #86769, #63647, #84902, #42752, #21453, #20051, #70272, #48932, #13898, #79233, #71669, #6803, #35676, #35192, #57912, #41817, #70728, #64591, #5861, #42285, #34731, #49409, #85840, #13438, #6324, #14375, #93416, #92469, #43235, #27635, #21930, #78299, #72133, #28115, #7249, #56534, #85391, #29025, #36125, #64120, #73515, #9549, #15280, #29504, #72579, #44137, #15751, #23771, #24227, #80594, #52184, #30413, #9075, #89078, #74420, #44611, #59304, #38436, #67345, #8624, #88152, #73042, #81516, #52636, #87686, #45518, #23311, #65500, #7701, #81065, #37501, #2475, #16210, #58843, #31352, #66410, #80140, #60240, #53104, #45061, #22839, #73961, #36586, #619, #58386, #14829, #87229, #22377, #43683, #1997, #37955, #1527, #30890, #16663, #51250, #59783, #8172, #66862, #37056, #65966, #1077, #29957, #88624, #51706, #46004, #17138, #2924, #54507, #69198, #83379, #61635, #47393, #75824, #4793, #82464, #17611, #90468, #67799, #82915, #81982, #61180, #3868, #54045, #18069, #62096, #25625, #46462, #18527, #24705, #33671, #90018, #11430, #68737, #54983, #68264, #31809, #40744, #76304, #74909, #46922, #76767, #75365, #60702, #10020, #10479, #10948, #90929, #91423, #39814, #40281, #32747, #4327, #62581, #47864, #33204, #26094, #11895, #69661, #83859, #19012, #39345, #26577, #38890, #25171, #89542, #53591, #3386, #32274, #93361, #42695, #79637, #64536, #7200, #70674, #28512, #14779, #12922, #56949, #43632, #34677, #49349, #48871, #72530, #14322, #36075, #72084, #42224, #50753, #78244, #49806, #5803, #20483, #92900, #43182, #41763, #13381, #7649, #64993, #36534, #71138, #6267, #21397, #85332, #65449, #85786, #96, #35621, #21881, #35135, #92415, #565, #50268, #77775, #13844, #29450, #64058, #63591, #27575, #28059, #78702, #57860, #58338, #20937, #86246, #57406, #28975, #87180, #56473, #71614, #79177, #6748, #86716, #44086, #8119, #80088, #1030, #29908, #72989, #58792, #37005, #22329, #51200, #15230, #65918, #48497, #33361, #69825, #39505, #91093, #77396, #75523, #25786, #12533, #3556, #18231, #17768, #41384, #76930, #4960, #40905, #11116, #19628, #47082, #18699, #68426, #83078, #61791, #12058, #10645, #75988, #70317, #33845, #5447, #39983, #68898, #90623, #34315, #69354, #4030, #63221, #92053, #55158, #54667, #26264, #32445, #61346, #90181, #56094, #25329, #54209, #46623, #62754, #62260, #47562, #91586, #26743, #32903, #55629, #27207, #84020, #83540, #76467 ),
 ( #11589, #84478, #40436, #4484, #19168, #48025, #21037, #72176, #191, #77877, #7292, #667, #64633, #27683, #36632, #13484, #5907, #86347, #36171, #48980, #20098, #34777, #57503, #65091, #21498, #93460, #50376, #78800, #7748, #85434, #20583, #28614, #70774, #85885, #84948, #64168, #6845, #57048, #49905, #29072, #79280, #49454, #14421, #56581, #65553, #93000, #43278, #71718, #57964, #71242, #63692, #43728, #86818, #13025, #13945, #79732, #78342, #92517, #41861, #42331, #42802, #21976, #29551, #35719, #50849, #14874, #72627, #6371, #35242, #28158, #9124, #24276, #82032, #59353, #38001, #22886, #31398, #67392, #37547, #89125, #66911, #15327, #22424, #2049, #52229, #53151, #74007, #16710, #80188, #30939, #17190, #51296, #66458, #46052, #44188, #58888, #58431, #74957, #23818, #45565, #81562, #51755, #60288, #87734, #88204, #73093, #30003, #8669, #52681, #8223, #80645, #10068, #74469, #38937, #15800, #44659, #1576, #67846, #16255, #73560, #2972, #87277, #59828, #30458, #88669, #37101, #66010, #1122, #23362, #81112, #2521, #45105, #9600, #38487, #82510, #89587, #76349, #25672, #62631, #47440, #83904, #53640, #11475, #91470, #24758, #39862, #26621, #17658, #32328, #31857, #55512, #90974, #19055, #55035, #25217, #33720, #61230, #32790, #46510, #3433, #75869, #26140, #75412, #90065, #84360, #47911, #19510, #54090, #82961, #10993, #48378, #83420, #18115, #77280, #12409, #69241, #68784, #40326, #10528, #39395, #68310, #70198, #46967, #3913, #60746, #76814, #4370, #61678, #11939, #40788, #90510, #69706, #41259, #33248, #54552, #18575, #62144, #4836, #6731, #86231, #63103, #34199, #19975, #71595, #21382, #35604, #78686, #64519, #92881, #21863, #5785, #34659, #13826, #84826, #6250, #5331, #78226, #20920, #71120, #35119, #79158, #42678, #63573, #93345, #41744, #50737, #13365, #28496, #85770, #72067, #85316, #48851, #57844, #57389, #91931, #64039, #80, #92399, #77756, #27086, #27559, #28043, #14306, #14763, #56933, #50252, #49789, #43166, #79621, #64977, #7184, #36059, #28958, #86698, #43617, #55973, #56454, #12905, #70657, #20465, #49332, #42206, #9013, #73447, #44544, #36988, #74356, #44995, #7633, #52572, #16143, #8557, #1927, #24160, #65900, #66346, #51639, #29892, #1460, #87618, #1012, #37892, #59718, #81916, #67279, #52118, #2409, #72972, #72513, #30346, #31289, #53040, #8101, #17068, #66797, #9479, #58776, #65433, #22769, #59236, #80525, #81000, #38365, #60175, #81452, #15678, #23709, #16600, #89013, #88082, #23238, #36518, #73896, #30821, #547, #88561, #45456, #29430, #58320, #87164, #22313, #51184, #80071, #15214, #44070, #17546, #11826, #75298, #18459, #83314, #40217, #89954, #39281, #69595, #9956, #61115, #2861, #69133, #11365, #38828, #90404, #18944, #10881, #84253, #45935, #46857, #10417, #47798, #40677, #67735, #31744, #18004, #47318, #3319, #75760, #54910, #25561, #76234, #60637, #33139, #76700, #82398, #39744, #68199, #90863, #4261, #74843, #53522, #89474, #62029, #33603, #24635, #25109, #46398, #54441, #32208, #83789, #26027, #62511, #4725, #68668, #91351, #26512, #53983, #3804, #55401, #32685, #82852, #61571, #35013, #85201, #20351, #93238, #27933, #19869, #85665, #55868, #35952, #27447, #42568, #6141, #86125, #5677, #62993, #71961, #20813, #48267, #78120, #14196, #48739, #34091, #77169, #77643, #49223, #28391, #28853, #13258, #56824, #63928, #13716, #93697, #79044, #42095, #92766, #43057, #7079, #71010, #49683, #12794, #21274, #57283, #92290, #50146, #78578, #70076, #12299, #71484, #6616, #64871, #35496, #64411, #41143, #57739, #19404, #5218, #56339, #91824, #26977, #41635, #84720, #70554, #34552, #63460, #16038, #79965, #88455, #22207, #87510, #14659, #58213, #36880, #52005, #50630, #87058, #52470, #73792, #74248, #51077, #15102, #65795, #9370, #44435, #43962, #16492, #45346, #30237, #905, #1354, #43514, #79520, #72412, #31183, #7528, #36413, #86584, #8908, #8452, #22657, #37785, #1820, #65329, #66692, #2300, #66239, #29321, #38254, #72861, #433, #87971, #30706, #7986, #21754, #29787, #59127, #59605, #23122, #80891, #44891, #80419, #67167, #58666, #51530, #23602, #15564, #73341, #37331, #81344, #67629, #4158, #32580, #76594, #33028, #32098, #39634, #18355, #88906, #25007, #11256, #89845, #17897, #54796, #75193, #90303, #61000, #53878, #24522, #61919, #61473, #24056, #40111, #3695, #82744, #83208, #11716, #53403, #46750, #39176, #17439, #75651, #10306, #82288, #25455, #47213, #69484, #83675, #68558, #18837, #60528, #60069, #10774, #47692, #40569, #89364, #4614, #54334, #90755, #46289, #52930, #68087, #76124, #3212, #69026, #25913, #81809, #16958, #45823, #74729, #9850, #38723, #2757, #31638, #71843, #85082, #49110, #33488, #91713, #34902, #41517, #56707, #85553, #77056, #62394, #20701, #33975, #12675, #5096, #93122, #62879, #6028, #70896, #27817, #77523, #26865, #57168, #91237, #48622, #84144, #49571, #92645, #26402, #78007, #6496, #92180, #55290, #19293, #34441, #55753, #35377, #28278, #48152, #12185, #5570, #63813, #84606, #63347, #42454, #13147, #78466, #41028, #13603, #64296, #69954, #27335, #19755, #71366, #86008, #70443, #56222, #20233, #21158, #50027, #41983, #78920, #14069, #42934, #23378, #66475, #38506, #89145, #17675, #2989, #81581, #31875, #7411, #6963, #9141, #60764, #53658, #36292, #82527, #2539, #10086, #88222, #93578, #52247, #59845, #1592, #16729, #38954, #67866, #82050, #30474, #53170, #17207, #89605, #30957, #38018, #46528, #88686, #23834, #35836, #59370, #9619, #16272, #31418, #60307, #50506, #64753, #24294, #81128, #45123, #72290, #24775, #74024, #74487, #45582, #46068, #66928, #2066, #28737, #57620, #52700, #86463, #74974, #67410, #21624, #79404, #14540, #43395, #19992, #75430, #76367, #39881, #77297, #41278, #3453, #39413, #47460, #47928, #32805, #11493, #84379, #26161, #19074, #32348, #62651, #12427, #18131, #40342, #68802, #26640, #76831, #10548, #82981, #61247, #11958, #63121, #68329, #54569, #46985, #83922, #75885, #19528, #40806, #91950, #48394, #69259, #55053, #33738, #90082, #4388, #55530, #33265, #62162, #70215, #90527, #69723, #90991, #4854, #3931, #5349, #91486, #25234, #34215, #27105, #55989, #84844, #54108, #61695, #11011, #25687, #83439, #18594, #13445, #92476, #62718, #77359, #27642, #56542, #33805, #12493, #91052, #5868, #41824, #12019, #63654, #41346, #83502, #90588, #70279, #26704, #85398, #48458, #84909, #54630, #5412, #20546, #25749, #40869, #49416, #18661, #33326, #32867, #78306, #92015, #20057, #56055, #26227, #34738, #62223, #91548, #47527, #4446, #76891, #27167, #76432, #55120, #42293, #48939, #71205, #83985, #19133, #69787, #61756, #84441, #47988, #11553, #40400, #34277, #4918, #63184, #69318, #55593, #19589, #77838, #12986, #70735, #44617, #87238, #21938, #36133, #22385, #15288, #92964, #51257, #15758, #79695, #42759, #51712, #28576, #21000, #7709, #80148, #64129, #35200, #49865, #72587, #44145, #36593, #14837, #65508, #153, #22845, #6810, #35684, #43690, #85847, #7257, #6332, #79242, #50810, #72141, #65050, #73050, #627, #64599, #29512, #71677, #80601, #14383, #58393, #86778, #8180, #86309, #78764, #58849, #37063, #28122, #29033, #1083, #93424, #13906, #57011, #57466, #57921, #65972, #21461, #29963 ),
 ( #50335, #43243, #87692, #89084, #9556, #60707, #82469, #66416, #89547, #82920, #53110, #16216, #25176, #2004, #88159, #74915, #24711, #37507, #8630, #23318, #46010, #53596, #10026, #81989, #38896, #67351, #90023, #73967, #9081, #17144, #59310, #74426, #73521, #52642, #24233, #45524, #38443, #17616, #67805, #37961, #2929, #45067, #54050, #81522, #31814, #60246, #46467, #59789, #52190, #32280, #75371, #1534, #2481, #68269, #66868, #81071, #30419, #30897, #31358, #10484, #18074, #39350, #3391, #61185, #88630, #23777, #16669, #76773, #91429, #12867, #70623, #47871, #26583, #11436, #19940, #55935, #26100, #77717, #55473, #3873, #10953, #84322, #40750, #41706, #62587, #5291, #68743, #19472, #5750, #39820, #54990, #34625, #32752, #47399, #46927, #63536, #12370, #34161, #70155, #40286, #48811, #76309, #11901, #61640, #48339, #75829, #69203, #77240, #83865, #63064, #91893, #90473, #25630, #27048, #4332, #19018, #18532, #92362, #33209, #41218, #84790, #27524, #90935, #62103, #56417, #54512, #69667, #83384, #85276, #4799, #33678, #64944, #87132, #79125, #58743, #20426, #21350, #78653, #22283, #80040, #42171, #78190, #86198, #86664, #71562, #50221, #29397, #45, #57813, #71085, #7598, #51155, #56899, #14272, #13793, #65402, #21828, #49295, #28006, #6217, #50703, #8066, #13328, #93313, #85738, #28925, #20884, #58289, #79591, #36956, #15181, #43132, #14732, #72483, #35086, #72037, #515, #7152, #36027, #44039, #35572, #43585, #36485, #72941, #42645, #65870, #978, #64005, #29859, #92843, #49756, #6697, #64486, #28463, #57357, #66766, #44965, #81418, #8983, #52086, #24129, #74808, #3282, #82362, #67247, #17511, #88050, #87586, #88529, #46363, #39246, #23206, #68162, #81882, #89439, #73865, #80493, #37862, #45423, #80969, #2377, #24597, #53486, #67701, #16114, #38797, #2829, #75264, #16568, #23677, #32175, #74323, #31712, #22731, #59686, #31255, #9447, #17037, #51605, #10379, #52543, #38333, #15641, #44510, #60142, #88981, #1897, #60604, #73416, #30788, #8526, #53007, #37405, #66315, #45903, #9924, #1430, #30314, #59203, #82815, #40638, #91787, #25074, #69098, #26938, #46819, #61538, #61076, #55826, #26474, #48227, #84215, #54405, #62953, #90370, #61991, #17966, #32650, #11328, #55363, #53947, #25526, #84682, #77129, #48698, #83278, #18422, #40179, #77603, #18908, #47282, #19831, #12753, #4686, #4225, #69557, #75721, #10844, #39708, #5643, #68632, #3765, #89918, #12259, #76661, #90826, #41103, #70033, #76199, #5176, #70516, #33560, #33101, #41594, #25986, #54871, #62470, #34050, #83752, #47763, #11788, #91312, #19363, #35914, #14155, #93656, #28354, #51040, #34977, #63891, #43020, #20316, #35458, #34518, #13681, #50106, #6580, #64376, #14618, #71923, #92726, #7044, #70973, #79927, #42532, #57700, #21237, #7489, #20775, #78080, #87020, #64832, #63425, #93202, #29281, #27898, #49186, #92254, #56787, #57244, #36374, #43475, #71443, #65287, #79001, #85163, #27411, #28816, #86086, #392, #86543, #21713, #56299, #50589, #58178, #13223, #79483, #22172, #42059, #85629, #6106, #15064, #72372, #43926, #72822, #49647, #78542, #37296, #8869, #29749, #73306, #51963, #67127, #65760, #8417, #67592, #88869, #89328, #66202, #1318, #80855, #24483, #59567, #30200, #31602, #60491, #45307, #16002, #16455, #58630, #870, #87471, #46252, #22618, #51493, #7947, #24018, #23567, #37747, #52892, #16921, #80381, #81771, #17404, #81309, #44397, #53362, #59090, #15522, #9331, #45779, #87932, #36842, #23083, #74212, #74690, #38213, #2263, #31145, #1781, #82248, #44854, #73757, #60032, #66655, #30665, #88417, #52434, #9814, #38687, #2722, #55254, #83635, #75614, #47657, #17860, #91678, #83168, #4577, #61884, #48117, #61436, #24968, #33938, #76558, #10268, #40074, #69917, #10738, #89805, #39138, #39595, #76084, #84109, #84569, #47175, #18798, #90716, #69447, #55718, #40994, #11216, #25876, #5055, #62845, #68991, #54758, #68517, #3653, #32544, #11681, #60954, #4121, #75156, #54296, #40531, #32993, #33452, #19259, #62354, #90267, #91195, #46711, #26830, #18319, #26363, #77020, #12149, #25418, #53843, #19716, #68049, #3176, #32060, #82709, #49072, #63312, #12631, #77971, #49538, #57587, #59323, #20666, #85974, #64261, #42895, #30432, #14509, #78432, #93091, #43365, #72261, #13569, #28245, #13113, #21590, #86431, #27778, #79372, #57132, #5534, #41477, #21124, #42419, #7378, #49992, #6930, #70409, #78887, #36259, #34405, #56672, #65179, #92143, #41949, #48587, #1549, #14034, #35803, #71808, #70862, #50469, #5993, #71331, #27298, #20193, #92608, #64716, #56185, #34866, #88175, #93543, #77487, #63779, #85521, #6461, #85044, #35335, #28702, #46939, #75841, #60720, #2494, #31829, #45080, #81085, #73980, #61651, #9097, #16229, #23334, #10497, #38909, #53123, #39366, #32296, #37974, #68282, #32763, #2943, #59802, #68755, #45538, #66882, #24729, #3404, #2020, #52203, #30912, #89559, #61201, #53611, #82482, #17629, #17160, #39832, #90037, #88643, #18085, #46481, #10964, #23791, #52655, #24249, #3886, #81535, #16683, #74439, #75384, #25189, #9571, #38458, #67364, #74928, #31371, #54062, #82933, #60260, #89097, #82003, #46025, #10039, #67818, #19484, #26594, #35096, #48350, #12383, #90484, #55005, #91905, #4810, #19951, #48822, #40299, #25642, #77729, #90947, #69679, #62116, #56426, #26111, #63075, #34173, #84801, #40761, #83877, #20437, #54525, #11912, #47412, #12879, #55946, #83394, #41229, #63545, #55484, #18544, #76321, #91443, #19028, #92374, #85288, #11447, #69214, #62601, #27059, #47882, #84333, #5761, #70169, #41717, #4343, #70633, #27533, #33220, #77253, #76786, #34634, #49306, #33690, #5303, #78200, #13339, #42180, #71093, #6226, #71572, #72493, #6708, #8079, #36497, #80505, #36967, #36038, #43597, #22293, #92854, #28937, #15191, #56, #21839, #58755, #79134, #524, #64955, #57823, #28474, #65880, #65414, #28017, #44051, #7609, #86674, #87143, #15653, #57367, #50715, #43143, #21361, #79601, #14283, #86209, #29409, #72047, #989, #49767, #64496, #64014, #29871, #58299, #51164, #80051, #50230, #87597, #93322, #14742, #85748, #35581, #7163, #72952, #56908, #22743, #51618, #44523, #73427, #8537, #20895, #78662, #13803, #42655, #8994, #61093, #89932, #74820, #16578, #45914, #59214, #1440, #88060, #75736, #23217, #30325, #37416, #24614, #53018, #67257, #53500, #46376, #52097, #82376, #46834, #17048, #73876, #82829, #59697, #80981, #38809, #17526, #16124, #66327, #44975, #9935, #75276, #67713, #2843, #31725, #31267, #53962, #37872, #66777, #60616, #1908, #38344, #30798, #45434, #81896, #9458, #2389, #10395, #89454, #88540, #39260, #23689, #17982, #74334, #68175, #24140, #3296, #52553, #81429, #25088, #32187, #60154, #88993, #26958, #18438, #61551, #68647, #47296, #54888, #70055, #12772, #83767, #62489, #69574, #84233, #41614, #55849, #18923, #4703, #91806, #84702, #47777, #33580, #76213, #34070, #5197, #90842, #62972, #91329, #32664, #39723, #26491, #76679, #19849, #55381, #48247, #90385, #19383, #48720, #3781, #10860, #77149, #4238, #25540, #11804, #40196, #77623, #54421, #11342, #69113, #33118, #83292, #62007, #26003, #40655, #12279, #41123, #18282, #2226, #31110, #10233, #81277, #2688, #1744, #74656, #17368 ),
 ( #11179, #67559, #39101, #46219, #89768, #76048, #61400, #31569, #75123, #90232, #25381, #60459, #68013, #59997, #68480, #10701, #9780, #32503, #3142, #52400, #59532, #32024, #89294, #54261, #60921, #53807, #23531, #24930, #83131, #88381, #38655, #47138, #16423, #88836, #30632, #40039, #82675, #17824, #46677, #23986, #3616, #52859, #24449, #45275, #67093, #45744, #75580, #74178, #81737, #9296, #39558, #38178, #16887, #53328, #82214, #85488, #26797, #40492, #92572, #27742, #12595, #48080, #77451, #90681, #32957, #25841, #13536, #54722, #61850, #68955, #56150, #84534, #5020, #85005, #77935, #83598, #20159, #19681, #27263, #18761, #48550, #5959, #47619, #76985, #34833, #76522, #69410, #4086, #63744, #34371, #49039, #92109, #62318, #70827, #4541, #69881, #11645, #33416, #19222, #63276, #91158, #26323, #56638, #13078, #20635, #55218, #84072, #12114, #49505, #55683, #40959, #78395, #33901, #41441, #62808, #70373, #91643, #5498, #41914, #80708, #93056, #35300, #42384, #29609, #58025, #72231, #58487, #51354, #64226, #87332, #51815, #22033, #78852, #87793, #64686, #57100, #43783, #22480, #6425, #71297, #85940, #14928, #80244, #72683, #50902, #7802, #36227, #58945, #42862, #71776, #79786, #28212, #43334, #21091, #21554, #86879, #14476, #7345, #15381, #36689, #6899, #65611, #14002, #22942, #50438, #723, #29129, #44245, #28670, #49961, #1179, #73155, #35773, #93512, #8278, #57555, #37158, #86400, #79341, #65145, #66067, #246, #30060, #53214, #31460, #10129, #90127, #75470, #45628, #60349, #10593, #39454, #16774, #89186, #74068, #82569, #24819, #88729, #46572, #24339, #66518, #73617, #82094, #9667, #68371, #3501, #74535, #17254, #32393, #61292, #38550, #46113, #9187, #17717, #53702, #23877, #25278, #75016, #1637, #8729, #38995, #67453, #54155, #67907, #3033, #37605, #31916, #15858, #30518, #52745, #44717, #59415, #16314, #88269, #23425, #60808, #89649, #52291, #38065, #81170, #45166, #2581, #66974, #2113, #59889, #31003, #81627, #83484, #48922, #70262, #70720, #47509, #18642, #33310, #5852, #40853, #54613, #12970, #41809, #26688, #62206, #91531, #11059, #47028, #39929, #27626, #68847, #75931, #83024, #5396, #4901, #19117, #34261, #91998, #3975, #63168, #92462, #62701, #25731, #34723, #11537, #32850, #84425, #27151, #61739, #18178, #90571, #55577, #56039, #19573, #48441, #77343, #76876, #63639, #76415, #40384, #12477, #69302, #83969, #4430, #91036, #33787, #55102, #47972, #84892, #41327, #26208, #20042, #12003, #69771, #77821, #79680, #43227, #29496, #42744, #6316, #15273, #29019, #85382, #65960, #7243, #64109, #57906, #20531, #56994, #57451, #65494, #1071, #28560, #138, #72127, #50796, #37048, #35668, #13890, #50319, #71660, #20983, #86761, #43677, #56525, #51244, #36119, #80133, #85832, #49400, #86293, #44131, #8165, #49850, #78291, #14823, #58379, #6793, #13429, #64583, #14367, #78749, #65036, #87223, #22370, #36580, #93408, #7695, #613, #21446, #73036, #42276, #71189, #21922, #72573, #35184, #79225, #92947, #28107, #53097, #81975, #73508, #29951, #17131, #30407, #9069, #1520, #89535, #59298, #2469, #67338, #24221, #73954, #23303, #53583, #87680, #45055, #80588, #45997, #89072, #22832, #74413, #2918, #88618, #58835, #51700, #30883, #88146, #31802, #24699, #15744, #44604, #1991, #31346, #81059, #59776, #38884, #9543, #60234, #8618, #74902, #60696, #66404, #23765, #52177, #10014, #67793, #37495, #16204, #37948, #17605, #46456, #66856, #81510, #16657, #38429, #45512, #75358, #10473, #39339, #41205, #69191, #76761, #55458, #32268, #62089, #48326, #33198, #54977, #91882, #18521, #33665, #4321, #90922, #61629, #5279, #69655, #61174, #77228, #40738, #26088, #26570, #48796, #90462, #83853, #91417, #34148, #83372, #90010, #47385, #19005, #32740, #11888, #63053, #27036, #12357, #25619, #70142, #55925, #47858, #84777, #19928, #41693, #4785, #62575, #3380, #54501, #84309, #11423, #19461, #77706, #46916, #25165, #12855, #3860, #76298, #68730, #54039, #40275, #82909, #18063, #75818, #10941, #39808, #502, #34612, #85726, #27508, #33, #36014, #63523, #21338, #43573, #35560, #15168, #70611, #71548, #35073, #72471, #36473, #92350, #56404, #42632, #43118, #27994, #6683, #79576, #50208, #14260, #85265, #57801, #7587, #13316, #64473, #63990, #21816, #72024, #5738, #78178, #20414, #7141, #58277, #49282, #49744, #42156, #79112, #71073, #14720, #64932, #87119, #65389, #93301, #28913, #86651, #6205, #28451, #50691, #57346, #86186, #29384, #20872, #22269, #51143, #80027, #92831, #56886, #78641, #13781, #24116, #81405, #73852, #67235, #89427, #8513, #8969, #23192, #1415, #37847, #59189, #37392, #74308, #31243, #53471, #38785, #23664, #67689, #73403, #44026, #44952, #2817, #24583, #66301, #82350, #65858, #8053, #966, #72926, #29845, #36945, #58728, #60130, #59673, #66753, #88969, #52996, #87573, #81870, #22717, #52530, #80478, #51592, #30302, #15628, #45409, #17021, #88035, #52073, #80956, #16554, #45890, #9434, #38321, #2365, #1881, #60592, #16100, #30774, #74795, #88516, #9912, #31699, #91661, #34388, #84551, #19698, #92591, #27280, #19241, #85024, #55236, #35318, #26814, #41933, #5518, #85505, #5038, #62337, #71313, #20176, #46351, #28228, #63293, #26343, #49056, #75252, #48098, #48567, #27760, #57116, #77470, #56167, #92126, #13095, #93074, #78414, #12613, #77952, #13553, #42402, #41458, #70844, #77002, #20652, #56656, #55700, #49522, #5977, #69428, #10367, #34850, #70390, #6443, #63761, #64243, #40509, #17498, #4559, #33433, #91177, #84091, #12131, #40977, #69899, #33918, #62827, #73176, #15398, #79356, #87810, #21571, #86895, #14018, #57572, #36243, #51371, #49976, #86415, #51833, #8295, #73636, #50454, #14491, #65161, #8747, #43799, #43349, #15879, #44735, #29626, #264, #741, #72246, #87349, #29147, #44265, #37176, #35788, #85956, #66084, #7361, #58043, #22049, #80726, #50918, #58504, #22498, #80262, #79802, #14944, #37624, #78868, #72699, #42878, #1196, #30077, #71791, #36708, #58962, #7818, #30534, #21108, #65629, #22959, #1654, #6913, #64701, #93527, #28686, #31935, #16792, #89205, #68388, #10147, #3051, #16333, #46590, #90145, #2131, #24357, #23895, #10613, #60826, #88287, #66994, #81187, #89670, #47047, #3992, #38568, #31020, #67927, #59907, #3520, #24838, #75948, #32411, #31479, #39013, #17735, #23442, #53232, #39471, #82115, #17273, #54173, #74556, #53721, #60367, #46131, #52764, #61309, #82588, #52310, #25295, #75488, #75034, #83042, #11079, #81645, #18195, #67470, #45646, #39947, #9686, #2599, #68863, #59436, #45183, #74085, #9204, #38082, #88749, #49986, #50930, #8758, #1666, #79367, #30548, #44279, #51844, #36254, #42889, #65173, #7832, #14503, #29637, #80739, #15890, #30090, #43360, #1208, #87822, #79814, #22972, #44746, #88298, #36720, #753, #78880, #22511, #7373, #14955, #73648, #58516, #87361, #6924, #37188, #37637, #21582, #43810, #72256, #66545, #51382, #14028, #57582, #71802, #80273, #59447, #35798, #29158, #50464, #15411, #278, #64711, #73187, #93538, #28697, #22061, #8306, #66096, #58055, #72710, #86906, #53247, #75046, #18208, #38579, #53733, #24369, #89218, #81657, #25306, #89683, #52321, #3531, #60840, #82129, #46600, #68874, #16805, #17286, #2613 ),
 ( #90158, #9698, #67007, #75962, #24850, #81199, #32879, #67940, #31032, #82599, #16345, #23907, #46143, #32421, #61767, #10158, #17746, #39027, #75501, #4004, #83054, #3063, #31948, #47058, #11092, #10623, #39481, #45661, #54184, #61320, #31491, #39958, #68402, #74098, #45195, #23455, #9217, #38097, #2143, #59921, #88761, #52778, #74569, #67482, #60379, #27658, #76443, #91069, #90600, #56556, #55133, #27182, #77851, #6344, #85410, #70293, #20558, #26240, #25760, #91560, #49430, #42308, #83997, #71217, #84922, #92490, #76904, #83516, #12034, #48471, #19145, #5424, #78318, #13457, #70748, #48000, #41837, #5882, #26717, #34752, #35216, #54643, #77371, #12508, #18673, #40881, #92027, #4933, #20073, #48953, #40412, #47539, #13001, #69799, #33820, #62235, #11564, #62730, #63197, #34289, #63667, #55604, #84453, #69330, #4461, #19603, #33338, #41359, #56069, #28134, #14849, #37075, #29044, #8641, #64143, #65066, #28589, #65984, #29976, #85861, #57023, #36145, #36605, #21472, #165, #73064, #43702, #7723, #21012, #51269, #1095, #6821, #57936, #57479, #15300, #65523, #92976, #71692, #49879, #641, #51723, #78777, #43254, #35695, #72601, #64609, #8194, #29525, #80615, #58860, #86791, #58405, #22397, #13918, #21950, #44159, #50823, #79707, #87706, #79254, #87251, #80162, #22857, #86320, #15771, #44630, #42775, #73532, #93435, #50349, #14395, #72152, #7268, #67362, #16681, #88641, #31369, #52653, #10037, #66428, #46937, #82001, #45078, #38907, #1547, #37972, #38456, #46479, #75839, #9568, #74926, #53121, #31827, #18083, #3402, #2492, #17157, #32293, #61199, #60258, #46023, #2017, #10495, #75382, #45536, #68280, #67816, #88172, #30430, #2941, #89095, #90035, #60718, #89557, #59321, #24726, #25187, #23332, #74437, #54060, #52201, #66880, #37518, #82931, #53609, #82480, #17627, #30910, #39364, #59800, #24247, #81083, #9095, #81533, #16227, #73978, #23789, #70631, #91903, #92371, #69212, #40297, #55002, #27531, #62597, #76319, #34632, #63543, #48348, #83875, #19482, #32761, #68753, #61649, #49303, #90482, #3884, #10962, #27057, #26592, #40759, #55944, #19949, #25640, #84799, #20435, #84331, #47409, #56424, #33218, #54523, #12380, #48820, #83392, #39829, #18542, #77251, #77726, #41227, #70166, #5301, #4808, #85285, #11445, #4341, #34171, #62114, #11910, #90945, #19026, #55482, #76784, #69677, #12877, #63073, #26109, #41715, #47880, #33688, #91441, #5758, #64953, #51162, #64494, #28015, #36965, #36036, #72950, #93320, #14740, #79132, #50228, #42652, #80049, #50713, #13337, #58297, #21837, #14280, #7607, #29869, #71570, #43141, #57365, #35579, #72045, #28472, #6705, #43595, #65412, #87595, #8077, #57821, #65878, #78660, #78198, #7161, #987, #58753, #13801, #22741, #72491, #15189, #86207, #71091, #21358, #54, #28935, #86672, #44049, #42178, #87141, #79599, #29406, #22291, #36495, #6224, #35094, #64012, #522, #92851, #56906, #85746, #20893, #49765, #74818, #9933, #1438, #51615, #38807, #52095, #30796, #23215, #17524, #80979, #24138, #88991, #45912, #1906, #44973, #75274, #15651, #66775, #8535, #67711, #17046, #44521, #2387, #24611, #16576, #89930, #80503, #52551, #16122, #53498, #46374, #73425, #37414, #23687, #53016, #8992, #81427, #60614, #31265, #81894, #66324, #2841, #82374, #88058, #45432, #73874, #31723, #89452, #30323, #59212, #37870, #10393, #39258, #59695, #88538, #74332, #60152, #9456, #68173, #3294, #32185, #61090, #38342, #67255, #77146, #53960, #83764, #70052, #54885, #83290, #26955, #84699, #46832, #82827, #90839, #91326, #76211, #18920, #34067, #69571, #62486, #75734, #12276, #55845, #61549, #47774, #18436, #5194, #26488, #17980, #32662, #10858, #55378, #12769, #63440, #4236, #90383, #33577, #25538, #62969, #84230, #41611, #91803, #26000, #4700, #41120, #39721, #76675, #19846, #11801, #40652, #48717, #40193, #19379, #48244, #77620, #47294, #70533, #5657, #68645, #34532, #25086, #3778, #54419, #11340, #69111, #33116, #62004, #49663, #86104, #13696, #56802, #28833, #79499, #7965, #87036, #71939, #22187, #92744, #92270, #93217, #51055, #43941, #27915, #72838, #86563, #411, #78558, #85182, #42548, #50123, #85644, #7060, #29298, #58193, #72389, #20792, #43493, #7506, #28369, #36391, #79943, #36859, #79021, #14174, #27427, #71463, #93675, #6596, #21732, #50608, #42074, #56317, #14635, #35474, #64391, #63909, #15081, #57261, #64848, #35930, #65304, #21253, #43037, #20331, #49201, #57717, #78097, #13238, #70990, #6122, #34992, #38703, #30683, #10285, #65775, #66670, #15541, #24499, #38232, #884, #75172, #16471, #73321, #67145, #29765, #66218, #1798, #74709, #58644, #37765, #9347, #81324, #60048, #46268, #31618, #59583, #45326, #60509, #89344, #88434, #74228, #30215, #67610, #9830, #44870, #2738, #2279, #22636, #87486, #31162, #23583, #53381, #88886, #24034, #51508, #52910, #82266, #80396, #73772, #17419, #44413, #1333, #8432, #37311, #81788, #16937, #45799, #59106, #87948, #23100, #52450, #51982, #80871, #16019, #8886, #3192, #39611, #5075, #26382, #26846, #3673, #68535, #83187, #55734, #90734, #10754, #62861, #91694, #76574, #18334, #47673, #60975, #32076, #89824, #77504, #24985, #53858, #39155, #55270, #54775, #69007, #84125, #48133, #82724, #19275, #48604, #18816, #75631, #84586, #61452, #17876, #40548, #77036, #46728, #68067, #32560, #11697, #12167, #69463, #4595, #33468, #33009, #19736, #90283, #25434, #62371, #54312, #40091, #47190, #76103, #83652, #11236, #4138, #41010, #91214, #61900, #69933, #25893, #33957, #20683, #37093, #660, #80636, #92625, #41966, #56689, #30451, #65545, #77989, #37539, #66450, #51288, #85536, #22416, #34422, #70426, #63329, #52222, #92160, #5552, #12651, #1114, #29544, #42437, #29995, #22878, #27317, #58880, #23355, #87270, #49091, #59344, #34885, #56203, #15318, #87726, #85062, #41496, #20213, #80180, #51744, #44178, #73084, #8215, #6478, #88195, #13130, #70879, #66002, #6010, #13585, #63796, #49554, #58424, #78449, #71347, #15792, #44651, #27796, #73552, #36624, #8661, #1568, #10518, #67838, #54081, #67383, #30931, #39852, #53632, #16248, #90501, #31849, #88662, #82502, #45098, #81555, #82023, #90055, #25661, #53143, #24749, #2963, #75404, #61669, #46958, #17180, #60738, #75860, #10983, #46044, #89579, #45558, #82951, #25208, #60280, #18105, #17650, #37994, #74000, #46501, #74949, #68775, #39387, #68302, #9117, #3423, #3904, #66902, #89117, #32781, #2041, #16703, #81105, #59821, #32318, #61221, #23811, #74459, #52674, #9591, #10059, #38479, #2513, #31390, #24268, #38929, #55025, #20455, #41735, #42197, #19046, #55963, #18564, #83895, #55503, #63563, #64030, #26612, #91922, #70188, #48840, #35110, #49323, #84352, #5322, #78217, #13356, #19501, #34190, #47902, #27550, #92390, #33709, #85306, #63094, #11466, #47430, #27077, #48368, #71110, #84817, #12897, #76340, #19966, #6241, #40317, #62621, #92871, #69232, #76804, #54543, #83411, #77745, #70648, #5776, #11930, #56444, #40778, #77271, #4361, #26130, #4826, #34650, #33238, #69697, #62134, #90965, #91461, #12400, #41247, #72059, #44536, #79613, #93337, #51630, #80516, #65425, #7176, #36510, #49781, #85762, #78677, #66338, #13818, #20912, #28034, #15205, #43609, #57836, #44063, #36980 ),
 ( #28488, #56923, #28950, #15668, #73439, #57381, #8549, #22305, #29884, #14297, #42670, #43158, #14754, #86224, #7624, #58768, #87610, #8092, #21374, #72964, #65892, #86689, #1004, #22758, #71587, #72505, #37429, #21854, #6723, #35596, #50729, #50244, #64511, #79149, #36051, #64969, #71, #538, #29422, #58312, #87156, #51176, #80063, #88074, #31281, #81909, #16135, #23701, #73888, #60167, #9471, #1452, #44987, #23229, #38356, #9949, #30337, #59710, #9005, #67271, #37884, #17061, #2401, #67728, #45926, #52564, #89005, #24153, #59228, #74348, #74836, #45447, #53032, #52110, #81444, #38821, #80993, #66789, #1919, #30812, #88553, #16592, #66180, #29728, #22150, #15501, #37726, #50564, #51018, #65264, #43452, #79905, #7467, #79461, #22596, #73283, #1757, #80830, #65736, #15981, #86522, #86064, #86998, #44833, #66632, #21687, #30644, #80360, #87911, #72349, #78979, #36350, #43903, #14595, #847, #23062, #51940, #1297, #370, #37274, #30179, #15043, #59063, #73736, #21214, #72800, #7924, #50084, #29256, #87450, #58152, #44372, #8396, #35893, #14131, #8848, #36815, #58609, #57679, #42996, #51471, #71902, #7022, #64811, #93635, #28792, #83144, #23544, #74668, #16435, #82688, #24943, #60009, #88849, #68028, #45287, #60471, #59543, #38667, #75136, #31582, #89306, #39572, #3155, #23998, #32038, #2239, #76062, #67571, #17838, #46232, #32517, #45758, #9309, #18295, #60933, #88393, #68968, #10246, #67105, #89780, #52414, #52871, #24462, #68494, #4098, #53341, #53820, #39115, #46690, #40051, #25394, #82226, #75592, #54274, #47153, #17380, #10715, #81750, #61413, #3629, #2700, #90245, #11191, #74190, #81289, #38191, #31123, #16900, #9792, #85020, #54735, #12609, #63757, #90693, #40973, #92587, #18774, #33429, #32969, #27756, #92122, #20172, #56163, #26339, #34846, #62333, #33914, #83613, #4555, #76998, #27276, #25853, #91173, #56652, #49052, #20648, #55232, #84087, #12127, #49518, #84547, #19237, #85501, #78410, #70386, #69895, #41454, #47632, #76536, #11658, #71309, #40505, #69424, #61862, #77947, #48563, #62823, #13091, #41929, #48094, #70840, #42398, #5514, #5034, #13549, #91657, #26810, #34384, #5973, #55696, #19694, #77466, #63289, #87345, #7814, #79798, #65625, #260, #22955, #29622, #51829, #64697, #36239, #79352, #57568, #29143, #21567, #93523, #36704, #22494, #15875, #1192, #14940, #30073, #6909, #6439, #7357, #58958, #80722, #35784, #44731, #737, #8291, #86411, #93070, #50450, #58039, #28682, #43795, #37172, #66080, #80258, #14487, #51367, #15394, #65157, #44261, #87806, #35314, #86891, #22045, #64239, #43345, #58500, #72242, #73172, #28224, #49972, #57112, #85952, #50914, #72695, #71787, #21104, #78864, #14014, #42874, #67923, #23891, #66989, #3515, #37620, #88745, #30530, #3047, #39009, #66531, #24353, #46586, #38564, #18191, #73632, #74551, #38078, #75484, #39467, #1650, #59432, #45642, #46127, #31016, #9682, #82584, #53228, #17269, #88283, #60822, #10609, #16329, #67466, #2127, #24834, #75030, #8743, #81183, #23438, #10143, #61305, #52306, #52760, #45179, #82110, #74081, #17731, #31931, #90141, #68384, #2595, #89665, #53717, #9200, #31475, #32407, #60363, #89201, #25291, #81641, #54169, #83038, #59903, #16788, #48934, #19585, #75944, #27163, #84437, #76887, #12015, #26222, #4442, #40865, #62219, #11549, #77355, #34273, #56537, #41820, #26700, #70731, #47523, #47043, #47984, #5864, #92472, #76428, #27638, #41341, #77834, #33322, #39943, #91048, #4914, #40396, #55589, #12982, #34734, #56051, #69314, #92011, #84905, #69783, #20053, #63650, #85394, #33800, #62714, #11074, #55116, #48454, #83981, #70275, #5408, #90584, #68859, #63180, #19129, #91544, #18656, #3988, #12489, #32863, #61752, #25745, #54626, #83498, #44139, #78302, #35679, #71200, #43686, #79690, #13441, #65045, #87231, #79236, #58845, #20542, #21456, #78760, #22379, #80142, #42288, #6327, #86304, #86772, #71672, #50329, #29506, #148, #57915, #35195, #7704, #51252, #57006, #14378, #13901, #65502, #21933, #49412, #28118, #64123, #50805, #8174, #92959, #93419, #85843, #29028, #20995, #58388, #14832, #37058, #15282, #43238, #72582, #36588, #49861, #72136, #621, #7252, #36128, #73044, #64594, #65968, #1079, #29959, #42755, #6806, #28571, #57461, #67801, #31354, #23773, #17140, #39347, #52186, #66864, #9551, #59785, #88626, #2926, #2477, #88154, #60242, #30415, #10481, #1999, #46006, #74422, #60704, #73963, #37503, #46464, #89080, #22841, #3388, #38438, #1529, #24229, #51708, #23313, #52638, #31811, #32276, #81518, #53106, #67347, #81984, #68266, #53593, #16665, #74911, #82466, #17613, #45520, #10022, #81067, #89544, #24707, #30892, #75367, #38892, #44613, #80596, #87688, #15753, #73517, #8626, #66412, #59306, #16212, #45063, #9077, #37957, #91890, #46924, #61637, #61182, #27044, #26580, #48336, #84318, #54509, #63061, #90470, #62099, #82917, #32749, #11432, #55469, #25173, #25627, #55932, #77237, #48807, #83381, #18529, #40283, #77714, #19015, #47395, #84787, #19937, #4796, #69200, #69664, #18071, #54047, #75826, #5747, #10950, #39816, #90020, #12367, #76770, #90932, #41215, #70152, #68739, #5288, #70620, #40747, #3870, #12864, #76306, #4329, #62584, #34158, #33206, #26097, #54986, #33675, #41703, #91426, #19469, #83862, #47867, #11898, #35083, #64002, #43129, #20423, #35569, #34622, #36482, #20881, #78187, #87129, #7149, #63532, #44035, #79122, #42167, #36024, #92359, #92840, #64483, #43582, #72937, #6694, #72034, #50218, #28922, #15177, #512, #93310, #14269, #29394, #58286, #28460, #64941, #28003, #65399, #72480, #13790, #22280, #42, #49292, #27521, #57810, #57354, #51152, #86661, #21825, #56414, #50700, #80036, #13325, #42642, #71082, #6214, #56896, #85735, #49753, #79588, #14729, #78650, #71559, #86195, #21347, #8980, #29856, #73413, #52083, #68510, #65867, #8523, #68984, #90261, #90708, #66312, #37402, #80966, #25869, #59683, #1427, #32986, #61877, #45420, #16111, #16565, #58740, #975, #87583, #47649, #22728, #51602, #8063, #25410, #23674, #37859, #54289, #18312, #80490, #83160, #18790, #81415, #44507, #54751, #30311, #15638, #10731, #47168, #59200, #88047, #23203, #74320, #76077, #39587, #3645, #32536, #1894, #83628, #44962, #73862, #61429, #66763, #30785, #88526, #52540, #11208, #40066, #4114, #56666, #85037, #77015, #49067, #19253, #93084, #84563, #5988, #63306, #42413, #12624, #27292, #71324, #6454, #77481, #56179, #69910, #49532, #85515, #55712, #13563, #20187, #33445, #40523, #77964, #70402, #35329, #92137, #34860, #4571, #13107, #64255, #69441, #19710, #28239, #62348, #12143, #76551, #57126, #41944, #63773, #92602, #5049, #78425, #33931, #41470, #91189, #48111, #26825, #70856, #26356, #62839, #85968, #27772, #21118, #91672, #48581, #5529, #11674, #34399, #20661, #55247, #84104, #72090, #13852, #43190, #56484, #92425, #85342, #72997, #49359, #27587, #34687, #21888, #50278, #64544, #50760, #43639, #78253, #79644, #44092, #14330, #71147, #80095, #56957, #13391, #36082, #14786, #42234, #63601, #6276, #7207, #72537, #65001, #103, #28982, #28520, #51206, #35145, #64068, #57868, #92908, #35629, #28068, #42705, #79186, #6756, #93370, #7656, #86724, #85794, #36541, #20945, #15236, #71623 ) ),
 .UNSPECIFIED., .F., .F., .F.,
 ( 4, 3, 3, 3, 3, 3, 3, 3, 3, 3, 3, 3, 4 ),
 ( 4, 3, 3, 3, 3, 3, 3, 3, 3, 3, 3, 3, 3, 3, 3, 3, 3, 3, 3, 3, 3, 3, 3, 3, 3, 3, 3, 3, 3, 3, 3, 3, 3, 3, 3, 3, 3, 3, 3, 3, 3, 3, 3, 3, 3, 3, 3, 3, 3, 3, 3, 3, 3, 3, 3, 3, 3, 3, 3, 3, 3, 3, 3, 3, 3, 3, 3, 3, 3, 3, 3, 3, 3, 3, 3, 3, 3, 3, 3, 3, 3, 3, 3, 3, 3, 3, 3, 3, 3, 3, 3, 3, 3, 3, 3, 3, 3, 3, 3, 3, 3, 3, 3, 3, 3, 3, 3, 3, 3, 3, 3, 3, 3, 3, 3, 3, 3, 3, 3, 3, 3, 3, 3, 3, 3, 3, 3, 3, 3, 3, 3, 3, 3, 3, 3, 3, 3, 3, 3, 3, 3, 3, 3, 3, 3, 3, 3, 3, 3, 3, 3, 3, 3, 3, 3, 3, 3, 3, 3, 3, 3, 3, 3, 3, 3, 3, 3, 3, 3, 3, 3, 3, 3, 3, 3, 3, 3, 3, 3, 3, 3, 3, 3, 3, 3, 3, 3, 3, 3, 3, 3, 3, 3, 3, 3, 3, 3, 3, 3, 3, 3, 3, 3, 3, 3, 3, 3, 3, 3, 3, 3, 3, 3, 3, 3, 3, 3, 3, 3, 3, 3, 3, 3, 3, 3, 3, 3, 3, 3, 3, 3, 3, 3, 3, 3, 3, 3, 3, 3, 3, 3, 3, 3, 3, 3, 3, 3, 3, 3, 3, 3, 3, 3, 3, 3, 3, 3, 3, 3, 3, 3, 3, 3, 3, 3, 3, 3, 3, 3, 3, 3, 3, 3, 3, 3, 3, 3, 3, 3, 3, 3, 3, 3, 3, 3, 3, 3, 3, 3, 3, 3, 3, 3, 3, 3, 3, 3, 3, 3, 4 ),
 ( 0.4999999999939828133, 0.5624999999954868324, 0.6249999999969908515, 0.6562499999977429166, 0.6874999999984949817, 0.7187499999992470467, 0.7499999999999990008, 0.7812500000007509549, 0.8125000000015030199, 0.8437500000022550850, 0.8750000000030071501, 0.9375000000045111692, 1.000000000006015188 ),
 ( -0.05833358852679956102, -0.001562739243874584211, -0.0006756947238288813938, 0.0002113497962168214232, 0.001985438836308227057, 0.005533616916491038325, 0.009081794996673850026, 0.01262997307685666086, 0.01440406211694806801, 0.01617815115703947343, 0.01972632923722228426, 0.02327450731740509510, 0.02682268539758790593, 0.02859677443767931135, 0.03037086347777071677, 0.03391904155795352760, 0.03746721963813633843, 0.04101539771831914927, 0.04278948675841055815, 0.04456357579850196010, 0.04811175387868477094, 0.05165993195886758177, 0.05520811003905039260, 0.05698219907914180149, 0.05875628811923321038, 0.06230446619941602121, 0.06585264427959883204, 0.06940082235978164982, 0.07117491139987305870, 0.07294900043996446759, 0.07649717852014727149, 0.08004535660033007538, 0.08359353468051289315, 0.08536762372060430204, 0.08714171276069571093, 0.09068989084087851482, 0.09423806892106131872, 0.09778624700124413649, 0.09956033604133554538, 0.1013344250814269543, 0.1048826031616097582, 0.1084307812417925621, 0.1119789593219753798, 0.1137530483620667887, 0.1155271374021581976, 0.1190753154823410015, 0.1226234935625238054, 0.1261716716427066232, 0.1279457606827980043, 0.1297198497228894132, 0.1332680278030722310, 0.1368162058832550487, 0.1403643839634378665, 0.1421384730035292754, 0.1439125620436206843, 0.1474607401238035020, 0.1510089182039863198, 0.1545570962841691098, 0.1563311853242604910, 0.1581052743643518999, 0.1616534524445347176, 0.1652016305247175354, 0.1687498086049003532, 0.1705238976449917621, 0.1722979866850831709, 0.1758461647652659887, 0.1793943428454488065, 0.1829425209256315965, 0.1847166099657229776, 0.1864906990058143865, 0.1900388770859972043, 0.1935870551661800221, 0.1971352332463628398, 0.1989093222864542487, 0.2006834113265456576, 0.2042315894067284754, 0.2077797674869112932, 0.2113279455670940832, 0.2131020346071854643, 0.2148761236472768732, 0.2184243017274596910, 0.2219724798076425087, 0.2255206578878253265, 0.2272947469279167354, 0.2290688359680081443, 0.2326170140481909621, 0.2361651921283737798, 0.2397133702085565699, 0.2414874592486479510, 0.2432615482887393599, 0.2468097263689221776, 0.2503579044491049954, 0.2539060825292878132, 0.2556801715693792221, 0.2574542606094706310, 0.2610024386896534487, 0.2645506167698362665, 0.2680987948500190843, 0.2698728838901104932, 0.2716469729302019021, 0.2751951510103847198, 0.2787433290905675376, 0.2822915071707502999, 0.2840655962108417087, 0.2858396852509330621, 0.2893878633311158799, 0.2929360414112986977, 0.2964842194914815154, 0.3000323975716643332, 0.3035805756518471510, 0.3071287537320299688, 0.3106769318122127865, 0.3142251098923956043, 0.3177732879725784221, 0.3213214660527612399, 0.3248696441329440576, 0.3284178222131268754, 0.3301919112532182843, 0.3319660002933096932, 0.3355141783734925109, 0.3390623564536752732, 0.3426105345338580355, 0.3443846235739494444, 0.3461587126140408532, 0.3497068906942236710, 0.3532550687744064888, 0.3568032468545893066, 0.3585773358946807154, 0.3603514249347721243, 0.3638996030149549421, 0.3674477810951377599, 0.3709959591753205776, 0.3727700482154119865, 0.3745441372555033954, 0.3780923153356862132, 0.3816404934158690310, 0.3851886714960518487, 0.3869627605361432576, 0.3887368495762346665, 0.3922850276564174843, 0.3958332057366002465, 0.3993813838167830088, 0.4011554728568744177, 0.4029295618969658266, 0.4064777399771486444, 0.4100259180573314621, 0.4135740961375142799, 0.4153481851776056888, 0.4171222742176970977, 0.4206704522978799154, 0.4242186303780627332, 0.4277668084582455510, 0.4295408974983369599, 0.4313149865384283688, 0.4348631646186111865, 0.4384113426987940043, 0.4419595207789768221, 0.4437336098190682310, 0.4455076988591596399, 0.4490558769393424576, 0.4526040550195252754, 0.4561522330997080932, 0.4579263221397995021, 0.4597004111798909110, 0.4632485892600737287, 0.4667967673402565465, 0.4703449454204393643, 0.4721190344605307732, 0.4738931235006221820, 0.4774413015808049998, 0.4809894796609877621, 0.4845376577411705243, 0.4863117467812619332, 0.4880858358213533421, 0.4916340139015361599, 0.4951821919817189777, 0.4987303700619017954, 0.5005044591019931488, 0.5022785481420846132, 0.5058267262222674310, 0.5093749043024502487, 0.5129230823826330665, 0.5146971714227244199, 0.5164712604628158843, 0.5200194385429987021, 0.5235676166231815198, 0.5271157947033643376, 0.5288898837434556910, 0.5306639727835471554, 0.5342121508637299732, 0.5377603289439127909, 0.5413085070240956087, 0.5430825960641869621, 0.5448566851042784265, 0.5484048631844612443, 0.5519530412646440620, 0.5555012193448268798, 0.5572753083849182332, 0.5590493974250096976, 0.5625975755051924043, 0.5661457535853752221, 0.5696939316655580399, 0.5714680207056493932, 0.5732421097457407466, 0.5767902878259235644, 0.5803384659061063822, 0.5838866439862891999, 0.5856607330263805533, 0.5874348220664720177, 0.5909830001466548355, 0.5945311782268376533, 0.5980793563070204710, 0.5998534453471118244, 0.6016275343872032888, 0.6051757124673861066, 0.6087238905475689243, 0.6122720686277517421, 0.6140461576678430955, 0.6158202467079345599, 0.6193684247881173777, 0.6229166028683001954, 0.6264647809484830132, 0.6282388699885743666, 0.6300129590286658310, 0.6335611371088486488, 0.6371093151890314665, 0.6406574932692142843, 0.6424315823093056377, 0.6442056713493971021, 0.6477538494295799198, 0.6513020275097627376, 0.6548502055899455554, 0.6566242946300369088, 0.6583983836701283732, 0.6619465617503111909, 0.6654947398304940087, 0.6690429179106768265, 0.6708170069507681799, 0.6725910959908596443, 0.6761392740710423510, 0.6796874521512251688, 0.6832356302314079866, 0.6850097192714993399, 0.6867838083115906933, 0.6903319863917735111, 0.6938801644719563289, 0.6974283425521391466, 0.6992024315922305000, 0.7009765206323219644, 0.7045246987125047822, 0.7080728767926875999, 0.7116210548728704177, 0.7133951439129617711, 0.7151692329530532355, 0.7187174110332360533, 0.7222655891134188710, 0.7258137671936016888, 0.7275878562336930422, 0.7293619452737845066, 0.7329101233539673244, 0.7364583014341501421, 0.7400064795143329599, 0.7417805685544243133, 0.7435546575945157777, 0.7471028356746985954, 0.7506510137548814132, 0.7541991918350642310, 0.7559732808751555844, 0.7577473699152470488, 0.7612955479954298665, 0.7648437260756126843, 0.7683919041557955021, 0.7701659931958868555, 0.7719400822359783199, 0.7754882603161611376, 0.7790364383963439554, 0.7825846164765267732, 0.7843587055166181266, 0.7861327945567095909, 0.7896809726368922977, 0.7932291507170751155, 0.7967773287972579332, 0.7985514178373492866, 0.8003255068774406400, 0.8038736849576234578, 0.8074218630378062755, 0.8109700411179890933, 0.8127441301580804467, 0.8145182191981719111, 0.8180663972783547289, 0.8216145753585375466, 0.8251627534387203644, 0.8269368424788117178, 0.8287109315189031822, 0.8322591095990860000, 0.8358072876792688177, 0.8393554657594516355, 0.8429036438396344533, 0.8464518219198172710, 0.8500000000000000888 ),
 .UNSPECIFIED. ) ;
#68541=CARTESIAN_POINT ( 'NONE',  ( -100.2162370998004661, -296.5324065943632945, -307.6733667738163831 ) ) ;
#68543=CARTESIAN_POINT ( 'NONE',  ( 34.80532095757826738, -292.4204426637509755, -284.3629331368638304 ) ) ;
#68544=CARTESIAN_POINT ( 'NONE',  ( 10.46917891676551093, -277.0633869961445157, -330.6572904885218804 ) ) ;
#68545=CARTESIAN_POINT ( 'NONE',  ( -0.5462705402492801232, -274.5558203383570230, -207.2981618509985253 ) ) ;
#68546=CARTESIAN_POINT ( 'NONE',  ( 37.33707448775041371, -274.2526925033810130, -252.8519235993141194 ) ) ;
#68548=CARTESIAN_POINT ( 'NONE',  ( -68.46841309576564072, -271.6430645188398785, -202.1114116155810052 ) ) ;
#68550=CARTESIAN_POINT ( 'NONE',  ( -65.37033610184988675, -296.8367015690104722, -341.4596994596136028 ) ) ;
#68554=CARTESIAN_POINT ( 'NONE',  ( -110.6996360347542776, -285.6244184340591801, -270.9253420812303261 ) ) ;
#68555=CARTESIAN_POINT ( 'NONE',  ( 36.21657354682313468, -283.5539769589865955, -289.4177281235543546 ) ) ;
#68556=CARTESIAN_POINT ( 'NONE',  ( -103.5743098842943226, -284.3193555158867980, -239.3035658067771010 ) ) ;
#68557=CARTESIAN_POINT ( 'NONE',  ( 17.10777756799823379, -274.6591231268566276, -320.1965719770602732 ) ) ;
#68558=CARTESIAN_POINT ( 'NONE',  ( 12.76761964058083088, -284.2044992727001045, -325.1326575853840382 ) ) ;
#68559=CARTESIAN_POINT ( 'NONE',  ( -51.43223250054848705, -275.7154883937388377, -342.6948213860720216 ) ) ;
#68561=CARTESIAN_POINT ( 'NONE',  ( 35.91155138593595808, -276.6837768033442444, -274.3156557491608964 ) ) ;
#68564=CARTESIAN_POINT ( 'NONE',  ( -114.0502448525816277, -279.4109720149994587, -265.8936817706091347 ) ) ;
#68567=CARTESIAN_POINT ( 'NONE',  ( -109.5017692797823514, -286.1170155089739069, -293.4956305377884291 ) ) ;
#68568=CARTESIAN_POINT ( 'NONE',  ( -97.32160743803765968, -295.1664816039354378, -312.2539866627246852 ) ) ;
#68569=CARTESIAN_POINT ( 'NONE',  ( -75.62014853386071422, -288.8976352219044088, -337.0549945700602734 ) ) ;
#68570=CARTESIAN_POINT ( 'NONE',  ( 2.783371771579112863, -285.1769438582871317, -208.6735704435149614 ) ) ;
#68571=CARTESIAN_POINT ( 'NONE',  ( -68.20357379545868071, -289.8810540651671772, -203.0752192651493999 ) ) ;
#68572=CARTESIAN_POINT ( 'NONE',  ( -69.16753041430311555, -284.6854772919191987, -336.5130849264336348 ) ) ;
#68573=CARTESIAN_POINT ( 'NONE',  ( 21.06697382105475214, -274.1995948486199381, -317.4284998610248749 ) ) ;
#68574=CARTESIAN_POINT ( 'NONE',  ( 7.447648527805312391, -286.8528826659853053, -332.0731907457429770 ) ) ;
#68575=CARTESIAN_POINT ( 'NONE',  ( -46.29274066174475166, -287.9387348557513633, -195.8971701904704332 ) ) ;
#68576=CARTESIAN_POINT ( 'NONE',  ( 25.61645148577000342, -284.9993870828843683, -229.2965399195133216 ) ) ;
#68578=CARTESIAN_POINT ( 'NONE',  ( -5.921152389044468833, -283.5699898319567751, -336.5274465075643207 ) ) ;
#68579=CARTESIAN_POINT ( 'NONE',  ( 6.877081978565874998, -290.4525920709832008, -331.2095906079471774 ) ) ;
#68582=CARTESIAN_POINT ( 'NONE',  ( -89.69635647249970134, -297.7033392421006397, -324.9152747110364885 ) ) ;
#68583=CARTESIAN_POINT ( 'NONE',  ( -66.83331135974327708, -277.6655957160806452, -201.3888194779807748 ) ) ;
#68584=CARTESIAN_POINT ( 'NONE',  ( -2.120726005228241284, -291.7035516898681067, -202.0555087003184838 ) ) ;
#68585=CARTESIAN_POINT ( 'NONE',  ( -109.9326886625786841, -294.7775098989829416, -283.7349414300272201 ) ) ;
#68586=CARTESIAN_POINT ( 'NONE',  ( 28.58610029905434047, -280.6754999593893558, -302.9537583182598723 ) ) ;
#68587=CARTESIAN_POINT ( 'NONE',  ( -36.69956105920720546, -272.1401272554613797, -195.9112232137441936 ) ) ;
#68588=CARTESIAN_POINT ( 'NONE',  ( -5.311542420477732840, -295.9367735326890738, -336.5211685940752204 ) ) ;
#68589=CARTESIAN_POINT ( 'NONE',  ( -37.37352853689063892, -300.5519495502701943, -195.3611179825600175 ) ) ;
#68590=CARTESIAN_POINT ( 'NONE',  ( -51.65143983541086214, -296.3523193208734483, -195.3543580251313188 ) ) ;
#68591=CARTESIAN_POINT ( 'NONE',  ( 10.54214184089140538, -292.6414439185925289, -329.4298554152745169 ) ) ;
#68593=CARTESIAN_POINT ( 'NONE',  ( -28.04979484130534217, -293.5975427623568521, -197.3097182586588190 ) ) ;
#68595=CARTESIAN_POINT ( 'NONE',  ( 35.78239982941985176, -294.3242115016623188, -268.0227998142505612 ) ) ;
#68597=CARTESIAN_POINT ( 'NONE',  ( -102.9966077819564845, -282.0806788966253862, -307.4511841741179410 ) ) ;
#68598=CARTESIAN_POINT ( 'NONE',  ( -36.99554865599080955, -295.0476662810420407, -343.3727214492190569 ) ) ;
#68599=CARTESIAN_POINT ( 'NONE',  ( 24.25510323288072456, -282.1671030528345909, -316.5653798607781937 ) ) ;
#68600=CARTESIAN_POINT ( 'NONE',  ( -98.03037258737450088, -283.5859558642252978, -317.7175254347922078 ) ) ;
#68601=CARTESIAN_POINT ( 'NONE',  ( -73.49076889010724756, -289.5716214850342567, -204.7798224669997751 ) ) ;
#68603=CARTESIAN_POINT ( 'NONE',  ( -0.7253004819445844076, -281.0547819986877016, -337.3232660508965068 ) ) ;
#68604=AXIS2_PLACEMENT_3D ( 'NONE', #11633, #53792, #32944 ) ;
#68605=CARTESIAN_POINT ( 'NONE',  ( -37.51474938202356668, -287.9745691729268628, -347.0648312298804967 ) ) ;
#68607=CARTESIAN_POINT ( 'NONE',  ( -15.33505475997019474, -296.3627373208905738, -340.8573922075017890 ) ) ;
#68608=CARTESIAN_POINT ( 'NONE',  ( 19.45150595521237946, -277.6767957354051077, -321.4995663681362998 ) ) ;
#68609=CARTESIAN_POINT ( 'NONE',  ( -109.1521241605427264, -278.3935030675257281, -257.1191208857741231 ) ) ;
#68610=CARTESIAN_POINT ( 'NONE',  ( -16.62865441239325293, -292.4792808192214579, -196.1993371135274344 ) ) ;
#68612=CARTESIAN_POINT ( 'NONE',  ( -106.9110606339439045, -282.2480116897767175, -299.9809707674999686 ) ) ;
#68614=CARTESIAN_POINT ( 'NONE',  ( -93.69086985602459094, -279.8646018496164629, -319.8562866529097732 ) ) ;
#68615=CARTESIAN_POINT ( 'NONE',  ( 33.87939142761410238, -292.3859421483160759, -253.2498223541569473 ) ) ;
#68616=CARTESIAN_POINT ( 'NONE',  ( -74.75941460635843328, -295.5543429864280824, -205.3021768647415399 ) ) ;
#68617=EDGE_LOOP ( 'NONE', ( #86827, #66401, #26961, #50807, #41203 ) ) ;
#68620=CARTESIAN_POINT ( 'NONE',  ( 35.59654044235114156, -292.9933352629919341, -265.3183356207289307 ) ) ;
#68622=CARTESIAN_POINT ( 'NONE',  ( -82.13390479932374433, -293.1952119285919025, -326.4764044574609443 ) ) ;
#68623=CARTESIAN_POINT ( 'NONE',  ( -34.04743167588155472, -297.1512035042145499, -193.5969219078835977 ) ) ;
#68624=CARTESIAN_POINT ( 'NONE',  ( -26.70633511247313052, -287.4997668309037522, -194.5439389313508514 ) ) ;
#68625=CARTESIAN_POINT ( 'NONE',  ( 28.22683077944572005, -287.8201497505969542, -302.4511126711154247 ) ) ;
#68626=CARTESIAN_POINT ( 'NONE',  ( -109.1576076481700284, -279.8555616938490971, -286.9452331251816304 ) ) ;
#68627=CARTESIAN_POINT ( 'NONE',  ( -68.49419641248647395, -299.3972907315938983, -203.2093744295884221 ) ) ;
#68629=CARTESIAN_POINT ( 'NONE',  ( -56.71970302032536182, -276.1023893226414430, -341.2067259695984376 ) ) ;
#68631=CARTESIAN_POINT ( 'NONE',  ( -113.5439911062901359, -272.5282768512489042, -258.9426176334921479 ) ) ;
#68632=CARTESIAN_POINT ( 'NONE',  ( -89.65602300256830404, -291.7171379959017941, -323.3188919055007204 ) ) ;
#68633=CARTESIAN_POINT ( 'NONE',  ( 28.88952403982315076, -295.6479434352949625, -308.1488594110221015 ) ) ;
#68635=CARTESIAN_POINT ( 'NONE',  ( -107.1013708393497268, -291.4932646068735949, -248.4675950932366959 ) ) ;
#68638=CARTESIAN_POINT ( 'NONE',  ( 25.48217255793715807, -291.1236033665029481, -227.9194496951986650 ) ) ;
#68639=CARTESIAN_POINT ( 'NONE',  ( -95.55789471610023611, -297.5666407242449623, -219.9166988193663315 ) ) ;
#68640=CARTESIAN_POINT ( 'NONE',  ( -86.11125958076856080, -297.0200338997015592, -216.0139234138655695 ) ) ;
#68643=CARTESIAN_POINT ( 'NONE',  ( -111.6465910024872983, -292.2914005872708572, -252.9976232931603306 ) ) ;
#68644=CARTESIAN_POINT ( 'NONE',  ( -2.659677404128715672, -294.9805209788416391, -198.2697987213421698 ) ) ;
#68645=CARTESIAN_POINT ( 'NONE',  ( -110.5072938928216502, -286.3493563833146140, -286.1325278324435999 ) ) ;
#68646=CARTESIAN_POINT ( 'NONE',  ( -0.8058290590329729719, -272.5383256362744646, -205.0382613768491069 ) ) ;
#68647=CARTESIAN_POINT ( 'NONE',  ( -16.25573009212761022, -276.2468732228163617, -198.9162276371535540 ) ) ;
#68648=CARTESIAN_POINT ( 'NONE',  ( 7.564001427921393628, -290.7501676547364582, -210.9911578786071686 ) ) ;
#68649=CARTESIAN_POINT ( 'NONE',  ( -112.8157320181750407, -280.5041551860678624, -263.1553515476312555 ) ) ;
#68650=CARTESIAN_POINT ( 'NONE',  ( -24.05509554437135478, -282.2265260481609630, -342.2454612465816126 ) ) ;
#68651=CARTESIAN_POINT ( 'NONE',  ( -73.93719678362836589, -278.6061805930011133, -337.7723650155444943 ) ) ;
#68652=CARTESIAN_POINT ( 'NONE',  ( 39.24431913614497347, -280.3059525514516395, -267.0897205644089922 ) ) ;
#68653=CARTESIAN_POINT ( 'NONE',  ( 195.1625751280944883, 283.5718810751147885, -110.6458996475216310 ) ) ;
#68654=CARTESIAN_POINT ( 'NONE',  ( 33.49179082183145084, -276.1144101630742966, -240.6360990762123038 ) ) ;
#68656=CARTESIAN_POINT ( 'NONE',  ( -21.51763337645937924, -275.7716244540266644, -195.7132334690824678 ) ) ;
#68657=CARTESIAN_POINT ( 'NONE',  ( 31.98288692825981272, -296.4805209788415823, -303.7098442033569654 ) ) ;
#68662=CARTESIAN_POINT ( 'NONE',  ( -66.43912295571479376, -290.5219125493131855, -337.7025482309915674 ) ) ;
#68663=CARTESIAN_POINT ( 'NONE',  ( 35.42161599284018081, -289.5912973851545189, -292.3032460647767721 ) ) ;
#68664=CARTESIAN_POINT ( 'NONE',  ( -82.61588540025805116, -289.0384784787281092, -327.7557241382404527 ) ) ;
#68665=CARTESIAN_POINT ( 'NONE',  ( 28.64899394918147024, -286.5423695688986641, -230.7013677973067729 ) ) ;
#68667=CARTESIAN_POINT ( 'NONE',  ( 35.82869930591363072, -279.8215298216422298, -260.3609744337043139 ) ) ;
#68668=CARTESIAN_POINT ( 'NONE',  ( 34.57946447596738437, -289.1732613046047504, -251.9193465711355202 ) ) ;
#68669=CARTESIAN_POINT ( 'NONE',  ( -53.86376685795306685, -281.7478142474320180, -342.2310316382112205 ) ) ;
#68671=CARTESIAN_POINT ( 'NONE',  ( -92.59015885009021929, -280.5545822504652733, -221.8770194202433572 ) ) ;
#68672=CARTESIAN_POINT ( 'NONE',  ( 36.46166604554806412, -288.2257441307552881, -249.0565273307610994 ) ) ;
#68674=CARTESIAN_POINT ( 'NONE',  ( -96.93225853203573195, -278.4544643727180073, -312.6552196315389551 ) ) ;
#68675=CARTESIAN_POINT ( 'NONE',  ( -99.69885131347328411, -289.9394640906909899, -225.8684847145223955 ) ) ;
#68676=CARTESIAN_POINT ( 'NONE',  ( -68.44478495440118593, -286.4566494713619136, -200.0847118230900890 ) ) ;
#68677=CARTESIAN_POINT ( 'NONE',  ( 5.140469346994207100, -287.1019880072113324, -206.1510190833839147 ) ) ;
#68678=CARTESIAN_POINT ( 'NONE',  ( -34.84441460484721631, -283.1866265158773217, -343.3308267492291179 ) ) ;
#68681=CARTESIAN_POINT ( 'NONE',  ( -113.1538831664231850, -292.4014177154692220, -271.2384846505107703 ) ) ;
#68683=CARTESIAN_POINT ( 'NONE',  ( 27.64239246561254149, -291.7042667578300552, -229.8831898257906232 ) ) ;
#68685=CARTESIAN_POINT ( 'NONE',  ( -34.01804562442430324, -273.1537256354559986, -197.2012808496322691 ) ) ;
#68686=CARTESIAN_POINT ( 'NONE',  ( -81.81951131364591845, -294.9887739415768806, -333.1560331110289894 ) ) ;
#68687=CARTESIAN_POINT ( 'NONE',  ( -60.45826189183085120, -290.2268603332114481, -200.3337824028981231 ) ) ;
#68688=CARTESIAN_POINT ( 'NONE',  ( -66.47233124773364921, -293.6788207533389823, -338.4006678459977024 ) ) ;
#68689=CARTESIAN_POINT ( 'NONE',  ( -110.1817003237764396, -291.6388122862322234, -279.3869074852918288 ) ) ;
#68692=CARTESIAN_POINT ( 'NONE',  ( 37.04155763170902560, -291.4088359899499778, -259.1870604028920297 ) ) ;
#68693=CARTESIAN_POINT ( 'NONE',  ( -66.46688798966675904, -297.4335620590681515, -339.5294755591189073 ) ) ;
#68694=CARTESIAN_POINT ( 'NONE',  ( 10.27732240190107404, -289.3177175755081976, -326.0684281963970079 ) ) ;
#68695=CARTESIAN_POINT ( 'NONE',  ( 2.650421355659904332, -278.4989863310857459, -334.2898925820521754 ) ) ;
#68696=CARTESIAN_POINT ( 'NONE',  ( -5.464077083346287722, -275.4369534850363266, -340.0161671107475740 ) ) ;
#68698=CARTESIAN_POINT ( 'NONE',  ( -3.488617787458530017, -297.6630494814447729, -193.5270647055053246 ) ) ;
#68699=CARTESIAN_POINT ( 'NONE',  ( 19.95197245330039948, -274.4465989728540194, -317.2362740257074734 ) ) ;
#68700=CARTESIAN_POINT ( 'NONE',  ( 5.776768445224250037, -278.7215219500786816, -209.6807104091703877 ) ) ;
#68701=CARTESIAN_POINT ( 'NONE',  ( 26.97713144978790467, -276.2755870676452901, -234.8968034778139611 ) ) ;
#68702=CARTESIAN_POINT ( 'NONE',  ( -104.2826161255517263, -276.4759916022910033, -306.7665321268673324 ) ) ;
#68704=CARTESIAN_POINT ( 'NONE',  ( -85.38338918329472449, -274.0190211939736287, -215.1947441740319391 ) ) ;
#68706=CARTESIAN_POINT ( 'NONE',  ( -0.1156751476317717242, -286.5799725893410823, -335.9382387648072950 ) ) ;
#68707=CARTESIAN_POINT ( 'NONE',  ( 11.54809790458018703, -274.5861260988357913, -216.0824656522480609 ) ) ;
#68708=CARTESIAN_POINT ( 'NONE',  ( 36.69122204383213415, -287.2846441276786322, -249.0027959762152818 ) ) ;
#68709=CARTESIAN_POINT ( 'NONE',  ( -37.28078186119692106, -300.0328001623263958, -195.0051416838755074 ) ) ;
#68710=CARTESIAN_POINT ( 'NONE',  ( -78.99072894804898226, -293.6145419364606823, -332.5959562351066552 ) ) ;
#68711=CARTESIAN_POINT ( 'NONE',  ( 37.38892614052306129, -280.9739934559451626, -288.2915573491141572 ) ) ;
#68713=CARTESIAN_POINT ( 'NONE',  ( -15.64921055647543113, -278.3325399754585305, -198.5133485269475102 ) ) ;
#68715=CARTESIAN_POINT ( 'NONE',  ( -109.8136088346350192, -289.1936160389217889, -282.0571966196503126 ) ) ;
#68718=CARTESIAN_POINT ( 'NONE',  ( -87.24119644184246170, -289.3570090168245201, -214.2998010148533581 ) ) ;
#68719=CARTESIAN_POINT ( 'NONE',  ( -35.39119581315596008, -275.5971646020306025, -196.6809751414244829 ) ) ;
#68720=CARTESIAN_POINT ( 'NONE',  ( 35.05668491798139996, -283.2894315467105457, -294.9608900034124304 ) ) ;
#68721=CARTESIAN_POINT ( 'NONE',  ( -109.6517776936459114, -270.9144871198463989, -248.2606236157619719 ) ) ;
#68722=CARTESIAN_POINT ( 'NONE',  ( -110.2282293906098403, -284.6167374029307098, -265.4652042273821166 ) ) ;
#68723=CARTESIAN_POINT ( 'NONE',  ( -16.49095269897191685, -275.7520711298907372, -199.7344720970027652 ) ) ;
#68724=CARTESIAN_POINT ( 'NONE',  ( -6.470121702911462158, -275.2711590382823488, -204.0320340672124360 ) ) ;
#68725=CARTESIAN_POINT ( 'NONE',  ( -35.91111981277754239, -285.0343997516923196, -345.3602532887544498 ) ) ;
#68726=CARTESIAN_POINT ( 'NONE',  ( -100.9792975836874263, -271.9702727400850790, -233.8656324821017165 ) ) ;
#68729=CARTESIAN_POINT ( 'NONE',  ( 38.06234131800047749, -293.1896170895284399, -254.7006362196658245 ) ) ;
#68730=CARTESIAN_POINT ( 'NONE',  ( -105.6075976347626550, -286.1346545762723395, -300.5540647970166219 ) ) ;
#68732=CARTESIAN_POINT ( 'NONE',  ( -37.37352853689063181, -274.5523547857346784, -350.3611179825600175 ) ) ;
#68733=CARTESIAN_POINT ( 'NONE',  ( -56.89283428102781670, -276.4951048376808558, -344.7256258353416456 ) ) ;
#68734=CARTESIAN_POINT ( 'NONE',  ( -109.6650790623762930, -289.2591196847549213, -246.2009382901833874 ) ) ;
#68735=CARTESIAN_POINT ( 'NONE',  ( -23.92040942575637885, -284.3977116968617338, -342.8219812576328422 ) ) ;
#68737=CARTESIAN_POINT ( 'NONE',  ( -68.44311413856341630, -279.2266082079889316, -337.5366208791062377 ) ) ;
#68738=CARTESIAN_POINT ( 'NONE',  ( -91.49826719089604410, -286.7245100815020464, -216.4568274653686331 ) ) ;
#68739=CARTESIAN_POINT ( 'NONE',  ( -39.79139435073248876, -282.0215683023473616, -195.3882684419180862 ) ) ;
#68740=CARTESIAN_POINT ( 'NONE',  ( 20.03445056607907304, -275.0216763594859231, -218.9312568692113530 ) ) ;
#68741=CARTESIAN_POINT ( 'NONE',  ( -74.09871668599650718, -277.3600304950582540, -338.0364611039502165 ) ) ;
#68743=CARTESIAN_POINT ( 'NONE',  ( -94.16610388149210564, -297.8018816038778027, -318.4672511339338143 ) ) ;
#68744=CIRCLE ( 'NONE', #70325, 6.338655513825452559 ) ;
#68747=CARTESIAN_POINT ( 'NONE',  ( -82.21955959476886733, -295.5871815227393995, -209.2526581300645319 ) ) ;
#68748=CARTESIAN_POINT ( 'NONE',  ( -109.5538390098064951, -277.9133885610037282, -281.4694679879060573 ) ) ;
#68749=CARTESIAN_POINT ( 'NONE',  ( 17.79308768683785047, -276.0245515724481038, -217.1045054658737854 ) ) ;
#68750=CARTESIAN_POINT ( 'NONE',  ( -33.20411764481407602, -287.8649705596163813, -196.4130114733624737 ) ) ;
#68751=CARTESIAN_POINT ( 'NONE',  ( -39.07253318013764698, -296.5936188479102498, -346.6481547039148836 ) ) ;
#68752=CARTESIAN_POINT ( 'NONE',  ( -101.2882926045836598, -297.1986598968338171, -312.6333417410305628 ) ) ;
#68753=CARTESIAN_POINT ( 'NONE',  ( -96.58092134334746959, -293.1802604321854346, -224.6364736401502284 ) ) ;
#68754=CARTESIAN_POINT ( 'NONE',  ( -71.76283344156870214, -277.5960702501733977, -203.8996020374821967 ) ) ;
#68755=CARTESIAN_POINT ( 'NONE',  ( 26.35606817054642192, -282.9511249409263769, -231.7397465992683863 ) ) ;
#68756=CARTESIAN_POINT ( 'NONE',  ( -109.5662562372726399, -294.8658824183827392, -252.2832526988492248 ) ) ;
#68757=CARTESIAN_POINT ( 'NONE',  ( -89.56923641862556451, -285.6388907345217376, -325.3200966539636738 ) ) ;
#68759=CARTESIAN_POINT ( 'NONE',  ( 17.12947347674059628, -285.7727784315820827, -221.2799912083861500 ) ) ;
#68760=CARTESIAN_POINT ( 'NONE',  ( -107.9785293115594556, -267.5055723263413370, -306.7646458841903723 ) ) ;
#68761=ORIENTED_EDGE ( 'NONE', *, *, #87140, .T. ) ;
#68762=CARTESIAN_POINT ( 'NONE',  ( -2.172475781232041658, -286.1976899962005518, -206.3105313853950236 ) ) ;
#68764=CARTESIAN_POINT ( 'NONE',  ( -27.39849985068416416, -284.0084369012947718, -346.4578404129265436 ) ) ;
#68765=CARTESIAN_POINT ( 'NONE',  ( -24.59691416342607084, -274.5524353766472245, -198.4091818242210650 ) ) ;
#68766=CARTESIAN_POINT ( 'NONE',  ( -7.483662960881081183, -285.2298117827686497, -199.7603914629277426 ) ) ;
#68767=CARTESIAN_POINT ( 'NONE',  ( 39.47492157886362207, -282.4878643230741204, -269.9196205137719744 ) ) ;
#68770=CARTESIAN_POINT ( 'NONE',  ( -84.15696897388352227, -280.9421669263935541, -210.0361406744585508 ) ) ;
#68771=CARTESIAN_POINT ( 'NONE',  ( 39.61932352314976669, -281.8440618636216755, -267.0540507914810178 ) ) ;
#68772=CARTESIAN_POINT ( 'NONE',  ( -6.998514795304330072, -286.1237833571631768, -333.4427485647536855 ) ) ;
#68773=CARTESIAN_POINT ( 'NONE',  ( 186.1196728968302807, 263.2780867284629380, -153.3933332796401317 ) ) ;
#68774=ORIENTED_EDGE ( 'NONE', *, *, #85141, .F. ) ;
#68775=CARTESIAN_POINT ( 'NONE',  ( 35.68787887162498862, -277.7632188463565512, -286.7507020004812262 ) ) ;
#68776=CARTESIAN_POINT ( 'NONE',  ( 196.5064352957230938, 285.3209794444068734, -111.6193314779800971 ) ) ;
#68777=CARTESIAN_POINT ( 'NONE',  ( 1.271917777350735523, -278.5902660704379059, -206.4198583178948070 ) ) ;
#68778=CARTESIAN_POINT ( 'NONE',  ( -3.789263988190406884, -294.2488211981072368, -202.1690061756827106 ) ) ;
#68779=CARTESIAN_POINT ( 'NONE',  ( -34.30525242549934006, -294.3615545954173172, -343.3999614411675338 ) ) ;
#68780=CARTESIAN_POINT ( 'NONE',  ( -111.5717673097279317, -290.3140031316360705, -250.0769123901437467 ) ) ;
#68782=CARTESIAN_POINT ( 'NONE',  ( -111.7363272031165877, -294.9064189675772809, -287.8546757928123156 ) ) ;
#68783=CARTESIAN_POINT ( 'NONE',  ( -0.6107764770033399238, -286.9556833610751028, -334.4299289185682937 ) ) ;
#68784=CARTESIAN_POINT ( 'NONE',  ( 34.84338867194817624, -295.1871566078384035, -252.9812277668234231 ) ) ;
#68785=CARTESIAN_POINT ( 'NONE',  ( -88.04676812577316980, -286.6396566742880623, -217.1611221501266300 ) ) ;
#68786=CARTESIAN_POINT ( 'NONE',  ( 39.00438816635619332, -294.5999787890484640, -278.8568824204251086 ) ) ;
#68787=CARTESIAN_POINT ( 'NONE',  ( -88.93330826803268963, -284.2932877703015606, -322.1650367118525082 ) ) ;
#68788=CARTESIAN_POINT ( 'NONE',  ( -66.78607382019364991, -294.2243742026189466, -341.0932623691219874 ) ) ;
#68789=CARTESIAN_POINT ( 'NONE',  ( -114.0895197921789475, -291.3082059912559316, -274.0935430447972294 ) ) ;
#68790=CARTESIAN_POINT ( 'NONE',  ( -53.38261371696017932, -292.3442006903745778, -195.0589653445444753 ) ) ;
#68791=CARTESIAN_POINT ( 'NONE',  ( -56.06354280048936545, -289.4666261606691364, -340.9721086161489438 ) ) ;
#68794=CARTESIAN_POINT ( 'NONE',  ( -98.11605028801338335, -299.0243104460866448, -225.0980612733765156 ) ) ;
#68795=CARTESIAN_POINT ( 'NONE',  ( -81.01136527582367819, -272.2688100568652203, -207.3606178859388649 ) ) ;
#68797=CARTESIAN_POINT ( 'NONE',  ( 18.15063361211283421, -279.9322721941948657, -222.5505533467530199 ) ) ;
#68800=CARTESIAN_POINT ( 'NONE',  ( 29.03968615844400247, -275.5665286336129043, -309.2589130072233274 ) ) ;
#68801=CARTESIAN_POINT ( 'NONE',  ( -104.3409500289874359, -295.4434811899757278, -239.5494696656958240 ) ) ;
#68802=CARTESIAN_POINT ( 'NONE',  ( -67.27943376017204002, -279.3093880613304805, -338.2919474162719098 ) ) ;
#68803=CARTESIAN_POINT ( 'NONE',  ( 36.87832963287976185, -273.6722593704744781, -268.8602316538309651 ) ) ;
#68804=CARTESIAN_POINT ( 'NONE',  ( -96.42905717839009583, -298.3643847634436952, -226.7989390556653007 ) ) ;
#68805=CARTESIAN_POINT ( 'NONE',  ( -109.6656366116340280, -297.4744831311123221, -282.3391931841145492 ) ) ;
#68807=CARTESIAN_POINT ( 'NONE',  ( -112.6026582454786791, -298.3040396182838663, -258.3523573068501378 ) ) ;
#68808=CARTESIAN_POINT ( 'NONE',  ( -102.7882370907312577, -271.0692105648158758, -232.9046508698549758 ) ) ;
#68809=CARTESIAN_POINT ( 'NONE',  ( 34.94004018409767554, -294.3517587600364891, -281.6104475441847512 ) ) ;
#68810=CARTESIAN_POINT ( 'NONE',  ( -5.772527946748679639, -291.0503147052444319, -203.8734514726233726 ) ) ;
#68811=CARTESIAN_POINT ( 'NONE',  ( 94.75641758632609424, -301.7060295618178429, -195.3160783195277475 ) ) ;
#68812=CARTESIAN_POINT ( 'NONE',  ( -5.145730870924443145, -274.9570345914210066, -200.4830351017815815 ) ) ;
#68813=CARTESIAN_POINT ( 'NONE',  ( -107.9406309504387309, -272.9663396913570068, -251.5987125653890075 ) ) ;
#68814=CARTESIAN_POINT ( 'NONE',  ( 33.76701217245756936, -283.2088181013708095, -245.2663396428328326 ) ) ;
#68815=CARTESIAN_POINT ( 'NONE',  ( -31.68953967179505327, -281.6670732206436583, -346.6720817301573447 ) ) ;
#68816=CARTESIAN_POINT ( 'NONE',  ( -25.79347455145516577, -276.2573182259811801, -346.3871087513002749 ) ) ;
#68818=CARTESIAN_POINT ( 'NONE',  ( -96.05743635781752232, -283.1384598110784623, -314.0081573595506939 ) ) ;
#68820=CARTESIAN_POINT ( 'NONE',  ( 36.98587463082740356, -279.4041693611255255, -258.8227859101094737 ) ) ;
#68821=CARTESIAN_POINT ( 'NONE',  ( 35.68852752380548310, -274.2506524425070893, -279.8199299924288539 ) ) ;
#68822=CARTESIAN_POINT ( 'NONE',  ( -105.7063685277205565, -280.9582691590790660, -239.3937158058713806 ) ) ;
#68825=CARTESIAN_POINT ( 'NONE',  ( -104.8902391374355432, -271.4130410592724729, -234.9819204281583040 ) ) ;
#68827=CARTESIAN_POINT ( 'NONE',  ( -110.3873860473396604, -280.3244698023506203, -288.1450483035851562 ) ) ;
#68828=CARTESIAN_POINT ( 'NONE',  ( 115.2448031289451222, -299.5541904835127980, -195.3611179825600175 ) ) ;
#68829=CARTESIAN_POINT ( 'NONE',  ( -80.71459139261448001, -285.5551912867497890, -332.2964514654198069 ) ) ;
#68831=CARTESIAN_POINT ( 'NONE',  ( -42.20800475863909895, -287.1133227628986333, -345.2158272255558131 ) ) ;
#68834=CARTESIAN_POINT ( 'NONE',  ( -107.8364880520261835, -295.6159085010800140, -249.9254780138570027 ) ) ;
#68835=CARTESIAN_POINT ( 'NONE',  ( -23.57903063128033949, -287.0141106076861206, -343.3619879842859746 ) ) ;
#68837=CARTESIAN_POINT ( 'NONE',  ( -87.41722264350329397, -295.3534229690173447, -214.5270540879756709 ) ) ;
#68838=CARTESIAN_POINT ( 'NONE',  ( -40.76580597458836053, -284.4898354643546554, -194.0795885639085441 ) ) ;
#68839=CARTESIAN_POINT ( 'NONE',  ( -8.958294350829858033, -282.0298461185421957, -202.2375340144853624 ) ) ;
#68840=CARTESIAN_POINT ( 'NONE',  ( 12.99255351634633548, -280.6007779521450516, -327.3559727052530661 ) ) ;
#68841=CARTESIAN_POINT ( 'NONE',  ( -29.17312194119513791, -288.9457509618566178, -342.9026531910508879 ) ) ;
#68842=CARTESIAN_POINT ( 'NONE',  ( -108.5472971228495709, -280.2213261818041019, -251.7336861317283194 ) ) ;
#68843=CARTESIAN_POINT ( 'NONE',  ( -81.39323883506125412, -280.2387028243218765, -211.8846254143956855 ) ) ;
#68844=CARTESIAN_POINT ( 'NONE',  ( 19.35243163830423896, -290.2184173490053354, -320.0210953710667923 ) ) ;
#68846=CARTESIAN_POINT ( 'NONE',  ( -44.04275839310808749, -273.9697827263126442, -193.5999494752568921 ) ) ;
#68847=CARTESIAN_POINT ( 'NONE',  ( -110.0349201090081408, -292.7515248190919124, -253.3482171182604930 ) ) ;
#68848=CARTESIAN_POINT ( 'NONE',  ( -111.2586520408596868, -298.6233781216987495, -305.9938812882205070 ) ) ;
#68849=ORIENTED_EDGE ( 'NONE', *, *, #2914, .T. ) ;
#68850=CARTESIAN_POINT ( 'NONE',  ( 35.11150258591253248, -273.8093906609569217, -290.4230913517876616 ) ) ;
#68851=CARTESIAN_POINT ( 'NONE',  ( 144.7857639756989272, -299.5541904835127980, -189.7068768330456123 ) ) ;
#68852=CARTESIAN_POINT ( 'NONE',  ( -94.98976197696771351, -294.2718370863009341, -320.1922466267114373 ) ) ;
#68853=CARTESIAN_POINT ( 'NONE',  ( -67.09140211203794024, -273.0001545457404291, -203.5728015461282325 ) ) ;
#68854=CARTESIAN_POINT ( 'NONE',  ( -72.67443622358190680, -291.0492125653405537, -335.0318649508368480 ) ) ;
#68855=CARTESIAN_POINT ( 'NONE',  ( -51.18576187134640776, -284.9915413161372157, -343.1204637525321459 ) ) ;
#68856=CARTESIAN_POINT ( 'NONE',  ( -92.40020871325489793, -292.7089727706038502, -217.3031190158896493 ) ) ;
#68857=CARTESIAN_POINT ( 'NONE',  ( 3.861746285214376240, -293.9092649499620507, -205.8345868115563633 ) ) ;
#68858=CARTESIAN_POINT ( 'NONE',  ( 33.95026548985166670, -293.1776144409390099, -254.6044039904427052 ) ) ;
#68859=CARTESIAN_POINT ( 'NONE',  ( -95.69373833104647531, -287.2010402676939975, -223.2234507385051074 ) ) ;
#68860=CARTESIAN_POINT ( 'NONE',  ( 15.75506794078392403, -282.4916337534894524, -326.1261000513601971 ) ) ;
#68861=CARTESIAN_POINT ( 'NONE',  ( -70.20412056124072819, -293.5615406150545255, -338.4148729281706096 ) ) ;
#68862=CARTESIAN_POINT ( 'NONE',  ( -95.33613207595536210, -283.7004270802664792, -321.0133229450572117 ) ) ;
#68863=CARTESIAN_POINT ( 'NONE',  ( 28.06590198351766219, -277.0502787984133874, -234.2855206176445790 ) ) ;
#68864=CARTESIAN_POINT ( 'NONE',  ( 17.40634833298267736, -290.6948066931273047, -313.9805196606274080 ) ) ;
#68865=CARTESIAN_POINT ( 'NONE',  ( -105.2489764546544819, -276.2515413668471638, -304.0784449347737564 ) ) ;
#68867=CARTESIAN_POINT ( 'NONE',  ( -40.24307391747935014, -282.5972550986023748, -343.3650252200162640 ) ) ;
#68868=CARTESIAN_POINT ( 'NONE',  ( -39.59105578060906794, -281.2295985340695097, -193.7782378419589975 ) ) ;
#68869=CARTESIAN_POINT ( 'NONE',  ( 36.91375762869408561, -286.8553261888745283, -289.8276843707673152 ) ) ;
#68870=CARTESIAN_POINT ( 'NONE',  ( -32.10769235822609602, -293.8791896603459577, -196.5202846107300445 ) ) ;
#68871=CARTESIAN_POINT ( 'NONE',  ( 22.03063201690669359, -277.7993008343123620, -318.1454180215478686 ) ) ;
#68872=CARTESIAN_POINT ( 'NONE',  ( 34.74201150433786012, -277.1947289564130301, -296.1540006689463667 ) ) ;
#68873=CARTESIAN_POINT ( 'NONE',  ( -72.84386188793519068, -277.3697397097414523, -334.1610509284795398 ) ) ;
#68874=CARTESIAN_POINT ( 'NONE',  ( -111.5231057501210472, -274.6391852789947166, -262.0565492657142386 ) ) ;
#68875=CARTESIAN_POINT ( 'NONE',  ( -111.4236459266276853, -282.6881124386372335, -259.7831345562686352 ) ) ;
#68876=CARTESIAN_POINT ( 'NONE',  ( -56.17950392809218130, -291.4827602418790207, -195.6678482789587292 ) ) ;
#68877=CARTESIAN_POINT ( 'NONE',  ( -9.832929372396007395, -290.2988956171479344, -341.4224150921079399 ) ) ;
#68878=CARTESIAN_POINT ( 'NONE',  ( 15.10623187868024075, -291.7338887116835053, -219.0688635841866869 ) ) ;
#68880=CARTESIAN_POINT ( 'NONE',  ( 31.66172632871591830, -291.7015746722387917, -237.4183817063719459 ) ) ;
#68881=CARTESIAN_POINT ( 'NONE',  ( -2.425592560932005259, -292.1942915473235303, -206.2146103394824195 ) ) ;
#68883=CARTESIAN_POINT ( 'NONE',  ( -7.029398635054750599, -289.7433279682696821, -340.8214298497816230 ) ) ;
#68884=CARTESIAN_POINT ( 'NONE',  ( -103.4655885512649292, -279.6255503964544005, -239.0728292689274497 ) ) ;
#68885=CARTESIAN_POINT ( 'NONE',  ( -107.4847219664850400, -295.8711797101441903, -239.2226317391341297 ) ) ;
#68886=CARTESIAN_POINT ( 'NONE',  ( -15.45042789957055973, -286.9795465448964933, -196.5895546472412718 ) ) ;
#68888=CARTESIAN_POINT ( 'NONE',  ( -12.71449119069791855, -286.6970519834939068, -197.4279645375964094 ) ) ;
#68889=CARTESIAN_POINT ( 'NONE',  ( -104.1309284958072112, -284.4883085933072948, -299.8786798860649014 ) ) ;
#68890=CARTESIAN_POINT ( 'NONE',  ( -104.4934034522946718, -256.0290196201358413, -326.6823371243384031 ) ) ;
#68891=CARTESIAN_POINT ( 'NONE',  ( 166.3698261927351894, 232.4625470284710218, -191.7400226694176695 ) ) ;
#68892=CARTESIAN_POINT ( 'NONE',  ( -111.6100336445428240, -270.6909421912098423, -270.3374203212270004 ) ) ;
#68893=CARTESIAN_POINT ( 'NONE',  ( 13.61643884026687168, -273.9857543381705796, -217.8647390635576073 ) ) ;
#68894=CARTESIAN_POINT ( 'NONE',  ( 34.67974540479879408, -274.2927788890602869, -256.6812986239779093 ) ) ;
#68895=CARTESIAN_POINT ( 'NONE',  ( -78.16449755504908126, -297.0263985776559252, -205.1458888302250330 ) ) ;
#68896=CARTESIAN_POINT ( 'NONE',  ( 180.6035871466845322, 251.0332377899103165, -164.5909838749037135 ) ) ;
#68897=CARTESIAN_POINT ( 'NONE',  ( 34.73072401280766996, -274.5648047631371469, -296.1855194985085404 ) ) ;
#68898=CARTESIAN_POINT ( 'NONE',  ( -83.84442522790524777, -275.1635020853752849, -212.7809949437168768 ) ) ;
#68900=CARTESIAN_POINT ( 'NONE',  ( -95.80102097273827155, -274.3038306074657839, -220.7021960780265886 ) ) ;
#68902=CARTESIAN_POINT ( 'NONE',  ( -108.4088176238139454, -290.8210112048931251, -287.3155643822057073 ) ) ;
#68903=CARTESIAN_POINT ( 'NONE',  ( -102.9723425791615483, -296.8320857822657786, -310.3208175766178556 ) ) ;
#68904=CARTESIAN_POINT ( 'NONE',  ( -100.7035475187257703, -297.6214020476631390, -226.6939116994128938 ) ) ;
#68905=CARTESIAN_POINT ( 'NONE',  ( -9.228919109890636463, -294.8407892609643568, -337.7443874408109536 ) ) ;
#68907=CARTESIAN_POINT ( 'NONE',  ( -97.63923743152092527, -279.8540450261616570, -315.9182779660990832 ) ) ;
#68910=CARTESIAN_POINT ( 'NONE',  ( -35.33134803361723186, -279.5843755276557658, -193.4357990271597316 ) ) ;
#68912=CARTESIAN_POINT ( 'NONE',  ( -48.63232638649421347, -278.1405619872154489, -342.7723992473208909 ) ) ;
#68913=CARTESIAN_POINT ( 'NONE',  ( 38.61729267791743325, -277.2863043842763204, -268.3104051183530601 ) ) ;
#68914=CARTESIAN_POINT ( 'NONE',  ( -112.7395859938250169, -276.5569796260549538, -271.5565909009673646 ) ) ;
#68915=CARTESIAN_POINT ( 'NONE',  ( -106.3665758327925630, -273.3627330007209366, -246.4121101625442236 ) ) ;
#68916=CARTESIAN_POINT ( 'NONE',  ( -108.6056013527174997, -271.2798114442667270, -251.3995940395351454 ) ) ;
#68917=CARTESIAN_POINT ( 'NONE',  ( -107.6188887331644253, -278.9804637243246361, -250.5634092380568063 ) ) ;
#68918=CARTESIAN_POINT ( 'NONE',  ( -9.756862339182497124, -287.3840636236464547, -341.7219965988486479 ) ) ;
#68919=CARTESIAN_POINT ( 'NONE',  ( -62.90011178328097685, -275.7195489672476469, -199.8503511327572539 ) ) ;
#68921=CARTESIAN_POINT ( 'NONE',  ( -100.4484019759146634, -289.2409949684019921, -307.4764043590747633 ) ) ;
#68923=CARTESIAN_POINT ( 'NONE',  ( -111.3955503567632803, -283.6407571029802170, -291.0816404924456151 ) ) ;
#68924=CARTESIAN_POINT ( 'NONE',  ( -1.963742169635317669, -280.8167700189771381, -335.3861727691576107 ) ) ;
#68925=CARTESIAN_POINT ( 'NONE',  ( 22.60393719647837329, -279.5354195512760498, -227.6774503367744842 ) ) ;
#68926=CARTESIAN_POINT ( 'NONE',  ( -70.60435852157448267, -283.6899729326881925, -203.7517825457707659 ) ) ;
#68927=CARTESIAN_POINT ( 'NONE',  ( 35.28611634801455921, -289.7933428701097114, -289.1253899940311385 ) ) ;
#68928=CARTESIAN_POINT ( 'NONE',  ( -105.6316608028370325, -279.3994312439810415, -297.2611509760015451 ) ) ;
#68929=CARTESIAN_POINT ( 'NONE',  ( -114.0438014563954710, -273.4268578562636662, -284.1485097187775182 ) ) ;
#68930=CARTESIAN_POINT ( 'NONE',  ( -71.29035959423477209, -293.6041527609718287, -203.4702246659599894 ) ) ;
#68931=CARTESIAN_POINT ( 'NONE',  ( -25.53070151702314661, -278.4405457324816098, -195.2979823992891113 ) ) ;
#68932=CARTESIAN_POINT ( 'NONE',  ( -69.28848268271894995, -278.1352935113894773, -336.1267475058205605 ) ) ;
#68933=CARTESIAN_POINT ( 'NONE',  ( -11.31240767397753899, -284.7141020944063143, -340.9324098505744587 ) ) ;
#68935=CARTESIAN_POINT ( 'NONE',  ( -40.25822760372736298, -291.0086644611014322, -345.8776510268894526 ) ) ;
#68936=CARTESIAN_POINT ( 'NONE',  ( -90.62632059579011923, -295.2973389989725774, -217.5088008853391557 ) ) ;
#68937=CARTESIAN_POINT ( 'NONE',  ( 24.57922159140330365, -286.1437314727256762, -224.8643238726434106 ) ) ;
#68938=CARTESIAN_POINT ( 'NONE',  ( -65.61480225624852380, -290.0760341272024903, -202.1780208905026655 ) ) ;
#68940=CARTESIAN_POINT ( 'NONE',  ( -18.90932575960783169, -275.4946553913699745, -341.5052748176499335 ) ) ;
#68941=CARTESIAN_POINT ( 'NONE',  ( -38.38298836310534767, -293.2049259984099194, -344.5890184130745979 ) ) ;
#68944=CARTESIAN_POINT ( 'NONE',  ( -58.72567299283868181, -290.2603453682210670, -197.1119988365325071 ) ) ;
#68945=CARTESIAN_POINT ( 'NONE',  ( -110.4071043827411245, -286.2878204282607726, -259.9742456721976396 ) ) ;
#68946=CARTESIAN_POINT ( 'NONE',  ( -77.61855095521517001, -287.8243273861113494, -334.8565760528361466 ) ) ;
#68947=CARTESIAN_POINT ( 'NONE',  ( -72.67272803051490371, -286.9999027482505198, -205.7937574203843667 ) ) ;
#68949=CARTESIAN_POINT ( 'NONE',  ( -67.62384642560651571, -286.4471729718327992, -203.7608676596886426 ) ) ;
#68950=CARTESIAN_POINT ( 'NONE',  ( 35.51295101858538317, -295.7783054081259024, -289.6122637093188246 ) ) ;
#68951=CARTESIAN_POINT ( 'NONE',  ( -110.4406884240068223, -276.3874328452529880, -289.5392829052302091 ) ) ;
#68952=CARTESIAN_POINT ( 'NONE',  ( 37.61334982015772255, -275.6654163587709263, -252.7685477816147284 ) ) ;
#68953=CARTESIAN_POINT ( 'NONE',  ( -7.731537073715645469, -290.5170120279115054, -200.8304994624267010 ) ) ;
#68954=CARTESIAN_POINT ( 'NONE',  ( -114.2320067192800934, -278.5007682141953183, -274.4697372532468762 ) ) ;
#68955=CARTESIAN_POINT ( 'NONE',  ( -110.1917356009836766, -298.3221409579185206, -286.6313097050213514 ) ) ;
#68958=CARTESIAN_POINT ( 'NONE',  ( -106.4258079636003487, -276.3344332384846780, -297.5319023446353981 ) ) ;
#68959=CARTESIAN_POINT ( 'NONE',  ( 24.64246932113718813, -278.9792107225019890, -228.0453069640036290 ) ) ;
#68961=CARTESIAN_POINT ( 'NONE',  ( -0.3643162538074650736, -273.0144120578602269, -203.5976188485319369 ) ) ;
#68963=CARTESIAN_POINT ( 'NONE',  ( -111.0775633625152352, -298.0574923514698185, -271.4929015331194933 ) ) ;
#68964=CARTESIAN_POINT ( 'NONE',  ( 29.48576758952929211, -280.9638427208157623, -308.0935365075171717 ) ) ;
#68965=CARTESIAN_POINT ( 'NONE',  ( -110.4478753724393272, -297.5505683042409828, -266.0142123389778703 ) ) ;
#68966=CARTESIAN_POINT ( 'NONE',  ( -111.7983145776895526, -298.0887743147670790, -252.7681978257350579 ) ) ;
#68967=CARTESIAN_POINT ( 'NONE',  ( -21.92542755902348972, -273.9219088088029253, -198.9858699847102343 ) ) ;
#68968=CARTESIAN_POINT ( 'NONE',  ( 35.23739184658464296, -295.3094169996229539, -251.4593704465850124 ) ) ;
#68969=CARTESIAN_POINT ( 'NONE',  ( 22.99056205213839021, -287.0783802454094484, -222.4964187186883748 ) ) ;
#68970=CARTESIAN_POINT ( 'NONE',  ( 38.38764741312459705, -273.7380947504636310, -274.0085121470153808 ) ) ;
#68971=CARTESIAN_POINT ( 'NONE',  ( -8.235099443345465176, -288.5147215272406243, -341.6621696271678843 ) ) ;
#68973=CARTESIAN_POINT ( 'NONE',  ( 35.68552585476193428, -286.6917875895680368, -276.5129934439735848 ) ) ;
#68974=CARTESIAN_POINT ( 'NONE',  ( -87.29786058700643991, -289.3554763249453003, -214.4202324127716111 ) ) ;
#68976=CARTESIAN_POINT ( 'NONE',  ( -45.58595926748305516, -157.7977398304416283, -369.2266198007532125 ) ) ;
#68977=CARTESIAN_POINT ( 'NONE',  ( -15.83951863778704983, -288.2741619087357208, -340.2398024371093470 ) ) ;
#68979=CARTESIAN_POINT ( 'NONE',  ( -94.21674153619659364, -284.7906799391855088, -321.9368889303878518 ) ) ;
#68980=CARTESIAN_POINT ( 'NONE',  ( 37.19636038565180058, -292.3805872585965062, -252.0063434334399233 ) ) ;
#68981=CARTESIAN_POINT ( 'NONE',  ( 23.10017023616907750, -282.5265307403540760, -223.9369996643913794 ) ) ;
#68982=CARTESIAN_POINT ( 'NONE',  ( 38.30453210848756385, -282.7189687946499816, -258.5748521250762337 ) ) ;
#68983=CARTESIAN_POINT ( 'NONE',  ( -90.74290821453503497, -283.6697172377529341, -320.1337106357008224 ) ) ;
#68984=CARTESIAN_POINT ( 'NONE',  ( -70.10265834386611061, -279.4838224160689037, -337.8417703598986463 ) ) ;
#68985=CARTESIAN_POINT ( 'NONE',  ( -105.2536086688994601, -297.0223986164335201, -233.9578916741046157 ) ) ;
#68986=CARTESIAN_POINT ( 'NONE',  ( -36.74880309919144850, -275.3749310985004399, -196.8578584263821369 ) ) ;
#68987=CARTESIAN_POINT ( 'NONE',  ( -105.5609628390411103, -288.1718896738771036, -300.7870317829269311 ) ) ;
#68988=CARTESIAN_POINT ( 'NONE',  ( -92.30538224948728043, -272.0383219201071938, -221.7182957665462482 ) ) ;
#68990=CARTESIAN_POINT ( 'NONE',  ( -112.3417001280813707, -270.0523547857346784, -270.3292895737545223 ) ) ;
#68991=CARTESIAN_POINT ( 'NONE',  ( -109.8218912173550592, -286.2521355777659551, -287.3854109486860580 ) ) ;
#68992=CARTESIAN_POINT ( 'NONE',  ( 24.64458364532417178, -295.2338065494631110, -315.5406699309430110 ) ) ;
#68993=CARTESIAN_POINT ( 'NONE',  ( -95.19202472406374227, -284.5749892476611649, -315.0719572128637083 ) ) ;
#68994=CARTESIAN_POINT ( 'NONE',  ( 31.63857023217360620, -275.0460832957413686, -304.1651247615131410 ) ) ;
#68995=CARTESIAN_POINT ( 'NONE',  ( -105.9169724211796932, -291.6534497624328424, -235.4479266698207311 ) ) ;
#68996=CARTESIAN_POINT ( 'NONE',  ( -112.3794791970542803, -282.5539312781099284, -281.2032826568294013 ) ) ;
#68997=CARTESIAN_POINT ( 'NONE',  ( 17.47156745347409768, -293.1422438658657939, -216.2374740188380713 ) ) ;
#68998=CARTESIAN_POINT ( 'NONE',  ( -109.8099774705498390, -290.7671582998805775, -279.3297447321289155 ) ) ;
#69001=CARTESIAN_POINT ( 'NONE',  ( -46.92665465413691095, -155.5347905584845876, -361.4716131824436047 ) ) ;
#69002=CARTESIAN_POINT ( 'NONE',  ( 23.71210760700578746, -283.6869792227523135, -316.1338207159045055 ) ) ;
#69003=CARTESIAN_POINT ( 'NONE',  ( -19.11405058567864046, -274.3380690714489560, -350.3683826091709648 ) ) ;
#69005=CARTESIAN_POINT ( 'NONE',  ( 35.82923101673086563, -280.4133757932644926, -265.8621282895097693 ) ) ;
#69006=CARTESIAN_POINT ( 'NONE',  ( 29.07556193523780053, -275.7255690293050066, -309.2775873942426870 ) ) ;
#69007=CARTESIAN_POINT ( 'NONE',  ( -60.32020819313539306, -281.7538362510173329, -199.0883761885025081 ) ) ;
#69008=CARTESIAN_POINT ( 'NONE',  ( 203.3621511278661558, 290.5486715743153923, -82.72705405358787800 ) ) ;
#69009=CARTESIAN_POINT ( 'NONE',  ( -87.94501165638187956, -282.3179127923633018, -327.6848262233436913 ) ) ;
#69010=CARTESIAN_POINT ( 'NONE',  ( -108.9773741398122979, -282.3002752627718905, -291.3872042961274929 ) ) ;
#69011=CARTESIAN_POINT ( 'NONE',  ( -30.61915173512961630, -299.8953510805454812, -194.3724624115683923 ) ) ;
#69012=CARTESIAN_POINT ( 'NONE',  ( -96.45451462719987035, -296.4438331992726603, -313.3203735610517242 ) ) ;
#69014=CARTESIAN_POINT ( 'NONE',  ( 35.20341932327453094, -292.0817637824853250, -258.5158738245784775 ) ) ;
#69015=CARTESIAN_POINT ( 'NONE',  ( 24.29093874842557454, -276.8161051338233847, -316.3473182172350562 ) ) ;
#69016=CARTESIAN_POINT ( 'NONE',  ( 23.79349837878535112, -274.9993523650677503, -230.4676660947376092 ) ) ;
#69017=CARTESIAN_POINT ( 'NONE',  ( 27.38054430966980846, -275.0149838859649094, -311.6000957578334010 ) ) ;
#69019=CARTESIAN_POINT ( 'NONE',  ( -91.93800927802118395, -271.2728727457489413, -218.9203180104351816 ) ) ;
#69022=CARTESIAN_POINT ( 'NONE',  ( 34.24522837432861166, -282.8393326364432028, -286.1578816472051017 ) ) ;
#69023=CARTESIAN_POINT ( 'NONE',  ( 1.594404928357462392, -284.2992462796009363, -335.6141158939761340 ) ) ;
#69024=CARTESIAN_POINT ( 'NONE',  ( -93.32782825662420123, -284.5673319346022367, -223.3563722043860196 ) ) ;
#69025=CARTESIAN_POINT ( 'NONE',  ( -69.61951093316086769, -275.8841165099086652, -336.7421432443401272 ) ) ;
#69026=CARTESIAN_POINT ( 'NONE',  ( 32.52502979169417330, -283.7429237958347699, -295.6031913031487761 ) ) ;
#69027=CARTESIAN_POINT ( 'NONE',  ( -48.73394337978491819, -275.6795843013470630, -343.2204453836848188 ) ) ;
#69028=CARTESIAN_POINT ( 'NONE',  ( 26.90081100285147642, -276.1502029206625934, -234.9406850904321402 ) ) ;
#69030=CARTESIAN_POINT ( 'NONE',  ( -113.9172619976245073, -279.2676864613799239, -277.3266344729814818 ) ) ;
#69035=CARTESIAN_POINT ( 'NONE',  ( -99.98873105979056675, -286.9846712174409049, -227.6578967912818143 ) ) ;
#69036=CARTESIAN_POINT ( 'NONE',  ( -84.59016397018206135, -294.9194389820477795, -326.2862533417253985 ) ) ;
#69038=CARTESIAN_POINT ( 'NONE',  ( -99.94323740639396192, -290.4930371838918859, -225.7028565169545402 ) ) ;
#69039=CARTESIAN_POINT ( 'NONE',  ( 36.00340951498611020, -285.6580138479193351, -260.0627904844827185 ) ) ;
#69040=CARTESIAN_POINT ( 'NONE',  ( 0.4870118026387388888, -285.1412635069577846, -207.1798879602125112 ) ) ;
#69041=CARTESIAN_POINT ( 'NONE',  ( -88.61667236855386420, -289.5611182563358170, -216.9156809169514588 ) ) ;
#69042=CARTESIAN_POINT ( 'NONE',  ( -110.3911967564691992, -285.8574363530156575, -262.7239055372378971 ) ) ;
#69043=CARTESIAN_POINT ( 'NONE',  ( 37.55865725566398083, -273.4907655324512348, -265.5929878854221329 ) ) ;
#69044=CARTESIAN_POINT ( 'NONE',  ( -15.62177554798462786, -284.7283674343338475, -197.2673661383413730 ) ) ;
#69045=CARTESIAN_POINT ( 'NONE',  ( -77.16271645649362654, -299.5185044682058901, -206.8057302778058215 ) ) ;
#69046=CARTESIAN_POINT ( 'NONE',  ( 28.53733591518565049, -285.0705969524191801, -234.0593931626272592 ) ) ;
#69047=CARTESIAN_POINT ( 'NONE',  ( 30.23400950511711827, -282.1159319646882864, -242.1311354273028087 ) ) ;
#69048=CARTESIAN_POINT ( 'NONE',  ( -90.28862254023624700, -291.7987423674472893, -323.7883355087533914 ) ) ;
#69051=CARTESIAN_POINT ( 'NONE',  ( -36.26987921769980261, -296.9589985929893032, -345.9263780219752675 ) ) ;
#69052=CARTESIAN_POINT ( 'NONE',  ( -8.454100406568541004, -278.4301387991229717, -201.1476277317395898 ) ) ;
#69053=CARTESIAN_POINT ( 'NONE',  ( -70.81810795460187080, -290.8188877708287805, -201.1983466351589982 ) ) ;
#69054=CARTESIAN_POINT ( 'NONE',  ( -93.70644615886274664, -294.2821684150115971, -318.0195078357724583 ) ) ;
#69055=CARTESIAN_POINT ( 'NONE',  ( 19.22634219515002485, -279.5758764286661631, -223.4235660725706509 ) ) ;
#69056=CARTESIAN_POINT ( 'NONE',  ( -18.89152418481160467, -272.3712197867750433, -198.1903506020499606 ) ) ;
#69057=CARTESIAN_POINT ( 'NONE',  ( 34.25965969912002151, -295.0850742414888259, -286.9843176487187861 ) ) ;
#69058=CARTESIAN_POINT ( 'NONE',  ( -37.37352853689063892, -288.5519495502701943, -195.3611179825600175 ) ) ;
#69059=CARTESIAN_POINT ( 'NONE',  ( -59.92426353831178432, -296.2447403286202530, -197.4175861963979628 ) ) ;
#69060=CARTESIAN_POINT ( 'NONE',  ( 38.69760079047769352, -291.7916543487301055, -270.3330041864758755 ) ) ;
#69061=CARTESIAN_POINT ( 'NONE',  ( -34.85540876630292217, -293.5092700483970134, -196.8138999951133599 ) ) ;
#69063=CARTESIAN_POINT ( 'NONE',  ( -41.61246328981560794, -292.7999642431800567, -197.2744426717202941 ) ) ;
#69065=CARTESIAN_POINT ( 'NONE',  ( -80.63759168149073275, -281.6557728833422516, -332.1001550752932303 ) ) ;
#69066=CARTESIAN_POINT ( 'NONE',  ( -61.01316628223349880, -295.3680104789256688, -339.4701896549527760 ) ) ;
#69067=CARTESIAN_POINT ( 'NONE',  ( -33.05874685161818860, -282.9996357027131353, -347.2550458299313050 ) ) ;
#69068=CARTESIAN_POINT ( 'NONE',  ( -114.3338800259359829, -284.1878073109184584, -272.8443154304382574 ) ) ;
#69070=CARTESIAN_POINT ( 'NONE',  ( -0.1006523332996065029, -286.5557158187147593, -335.3294033923898496 ) ) ;
#69072=CARTESIAN_POINT ( 'NONE',  ( 23.68882309526330232, -280.6472268829167547, -316.1648622569413192 ) ) ;
#69073=CARTESIAN_POINT ( 'NONE',  ( 22.15658761977326208, -287.1245137316765295, -318.7702737150486314 ) ) ;
#69074=LINE ( 'NONE', #74296, #3728 ) ;
#69075=CARTESIAN_POINT ( 'NONE',  ( 8.743457688748675238, -296.0087700457601159, -328.0687969812492497 ) ) ;
#69076=CARTESIAN_POINT ( 'NONE',  ( -39.92471464559405092, -278.5092423588239967, -346.7411867980971465 ) ) ;
#69077=CARTESIAN_POINT ( 'NONE',  ( -9.235287070782970176, -280.0967488616905143, -202.9658879445917989 ) ) ;
#69078=CARTESIAN_POINT ( 'NONE',  ( -36.38050047534928666, -292.2305704265120880, -193.3540852250272621 ) ) ;
#69079=CARTESIAN_POINT ( 'NONE',  ( -31.76738481394369984, -281.0621908106563183, -345.7282432126794447 ) ) ;
#69080=CARTESIAN_POINT ( 'NONE',  ( 23.12049151693259219, -293.1851431141279249, -311.7744914200487756 ) ) ;
#69081=CARTESIAN_POINT ( 'NONE',  ( -104.7054917506405332, -294.9866993951073937, -237.3896117407235806 ) ) ;
#69083=CARTESIAN_POINT ( 'NONE',  ( 132.9888089158688445, -299.5541904835127980, -188.7117359724263679 ) ) ;
#69084=CARTESIAN_POINT ( 'NONE',  ( 12.39217848628290497, -293.8448432859474906, -323.9517551571413492 ) ) ;
#69086=CARTESIAN_POINT ( 'NONE',  ( 27.33386217378598815, -285.4809262143061801, -301.5434626090942629 ) ) ;
#69087=CARTESIAN_POINT ( 'NONE',  ( -96.80459177145193905, -272.4042928292710144, -221.6751666727004988 ) ) ;
#69088=CARTESIAN_POINT ( 'NONE',  ( 22.78181160526299109, -279.0665462617046728, -224.2371088011632878 ) ) ;
#69091=CARTESIAN_POINT ( 'NONE',  ( -18.32092974086830495, -287.6073113321486403, -196.2016579321515053 ) ) ;
#69092=CARTESIAN_POINT ( 'NONE',  ( -63.82287437146379006, -289.2404807025203013, -338.4428526538401343 ) ) ;
#69093=CARTESIAN_POINT ( 'NONE',  ( -51.39431815137975690, -278.7552430099216281, -342.7021967504224449 ) ) ;
#69094=CARTESIAN_POINT ( 'NONE',  ( -69.72080305854845506, -299.3799733593133396, -203.8061203483416080 ) ) ;
#69095=CARTESIAN_POINT ( 'NONE',  ( -93.92188349220010934, -276.6877070892334700, -317.1334981513923026 ) ) ;
#69097=CARTESIAN_POINT ( 'NONE',  ( -51.79248209061327657, -297.5389691031875827, -194.6964827588738842 ) ) ;
#69098=CARTESIAN_POINT ( 'NONE',  ( -108.7840730191190204, -292.7441415099378332, -249.4040483788558049 ) ) ;
#69099=CARTESIAN_POINT ( 'NONE',  ( 34.73641292525844193, -295.4689581511520942, -295.2451178575328754 ) ) ;
#69101=CARTESIAN_POINT ( 'NONE',  ( -71.21263066397611396, -290.1630777622050346, -335.1568366519673532 ) ) ;
#69104=CARTESIAN_POINT ( 'NONE',  ( -109.7576627626421413, -297.5305448026135764, -244.4914225431175794 ) ) ;
#69105=CARTESIAN_POINT ( 'NONE',  ( -93.77518860890138797, -289.3887018914161899, -219.8085032185672958 ) ) ;
#69106=CARTESIAN_POINT ( 'NONE',  ( -85.20658848613682324, -297.7446641055990995, -210.0726717104436716 ) ) ;
#69109=CARTESIAN_POINT ( 'NONE',  ( -96.93434827407746468, -292.7164318225183024, -222.7016588705756419 ) ) ;
#69110=CARTESIAN_POINT ( 'NONE',  ( -55.56934967048406548, -291.7662352645559167, -350.3683826091709648 ) ) ;
#69111=CARTESIAN_POINT ( 'NONE',  ( -107.8938622612846956, -286.2266261901499433, -295.4636370617670877 ) ) ;
#69112=CARTESIAN_POINT ( 'NONE',  ( 22.97358053910587472, -272.9466195794827286, -226.0655725294749629 ) ) ;
#69113=CARTESIAN_POINT ( 'NONE',  ( -99.05035829400321745, -275.0408417615836925, -228.6355270060332145 ) ) ;
#69114=CARTESIAN_POINT ( 'NONE',  ( -106.4590179936268157, -288.2675733135411065, -298.1421274133592192 ) ) ;
#69115=CARTESIAN_POINT ( 'NONE',  ( -107.5035164782560742, -280.0434765697297053, -298.9552608214577845 ) ) ;
#69116=CARTESIAN_POINT ( 'NONE',  ( -35.66279932563350030, -280.0737646465173043, -197.3680239662895701 ) ) ;
#69117=CARTESIAN_POINT ( 'NONE',  ( 17.14431727601325761, -280.2044743842694174, -221.6254372569278246 ) ) ;
#69118=CARTESIAN_POINT ( 'NONE',  ( 35.77210784752028871, -276.9239420079633192, -293.5098456583690449 ) ) ;
#69119=CARTESIAN_POINT ( 'NONE',  ( 12.74419818758856060, -279.5279127641941272, -212.4006874507052203 ) ) ;
#69120=CARTESIAN_POINT ( 'NONE',  ( 187.5249191740372225, 269.5786286523873514, -137.8896985354353149 ) ) ;
#69121=CARTESIAN_POINT ( 'NONE',  ( 2.286242977736494986, -275.5106964986985645, -204.6158037921495350 ) ) ;
#69123=CARTESIAN_POINT ( 'NONE',  ( 0.8316525005456222308, -276.0717705733681555, -204.2740200279934299 ) ) ;
#69124=CARTESIAN_POINT ( 'NONE',  ( -37.37352853689063892, -300.5519495502701943, -195.3611179825600175 ) ) ;
#69127=CARTESIAN_POINT ( 'NONE',  ( 31.69510081755798936, -288.9587866717197926, -295.0217381787643376 ) ) ;
#69128=CARTESIAN_POINT ( 'NONE',  ( 30.78892748424178905, -289.7517901133387568, -304.1279118552374143 ) ) ;
#69129=CARTESIAN_POINT ( 'NONE',  ( -92.49408472459907671, -289.2169206684125697, -318.4170538630988290 ) ) ;
#69130=CARTESIAN_POINT ( 'NONE',  ( -0.9930908772130121465, -286.0291765328881866, -202.5503112560963359 ) ) ;
#69132=CARTESIAN_POINT ( 'NONE',  ( 19.09309330472423838, -280.6204841067794860, -317.9365322202862671 ) ) ;
#69133=CARTESIAN_POINT ( 'NONE',  ( -2.770378220405110170, -290.4508535341478819, -336.1119664927302324 ) ) ;
#69134=CARTESIAN_POINT ( 'NONE',  ( -81.05280504165224897, -282.1375520136339219, -329.7546028229263015 ) ) ;
#69135=CARTESIAN_POINT ( 'NONE',  ( -106.9169831515794158, -280.1816977288369799, -246.5293538906025503 ) ) ;
#69136=CARTESIAN_POINT ( 'NONE',  ( -78.66164416873338894, -278.1174831519164172, -330.6775999518185358 ) ) ;
#69137=CARTESIAN_POINT ( 'NONE',  ( -96.99060916388398823, -288.6992586151886826, -318.4444385517433602 ) ) ;
#69138=CARTESIAN_POINT ( 'NONE',  ( -114.1656263199322439, -285.3954601322072904, -267.1314136815969960 ) ) ;
#69139=CARTESIAN_POINT ( 'NONE',  ( -87.71438949609948565, -285.8630994426134748, -212.1345925866928610 ) ) ;
#69140=CARTESIAN_POINT ( 'NONE',  ( -2.426796353345956891, -282.7432800014123586, -334.4842952976615038 ) ) ;
#69143=CARTESIAN_POINT ( 'NONE',  ( -100.6648485274051126, -292.9693778453632831, -228.6678392213815698 ) ) ;
#69144=CARTESIAN_POINT ( 'NONE',  ( -16.74318851087497961, -290.9976653230809802, -196.6793726809117970 ) ) ;
#69145=CARTESIAN_POINT ( 'NONE',  ( -1.597347459022061766, -273.5970631480266775, -206.4268879460287280 ) ) ;
#69146=CARTESIAN_POINT ( 'NONE',  ( -47.62616119627649880, -294.5282284634277516, -346.5683528550601977 ) ) ;
#69147=CARTESIAN_POINT ( 'NONE',  ( -91.25332714646035015, -289.7478700355291039, -220.1006087151738200 ) ) ;
#69148=CARTESIAN_POINT ( 'NONE',  ( 6.647455419184660208, -292.6850485722981148, -329.9474766471125236 ) ) ;
#69149=CARTESIAN_POINT ( 'NONE',  ( -66.47258166540430580, -290.6472966164407126, -337.7839770994312403 ) ) ;
#69151=CARTESIAN_POINT ( 'NONE',  ( -108.5405455545936064, -292.8588280645182067, -246.6246022097248272 ) ) ;
#69152=CARTESIAN_POINT ( 'NONE',  ( 19.93051215466206116, -290.8794933480363056, -221.6595997707165111 ) ) ;
#69153=CARTESIAN_POINT ( 'NONE',  ( 32.25513783405078527, -295.9180969805728978, -298.4493555469398416 ) ) ;
#69154=CARTESIAN_POINT ( 'NONE',  ( 23.72365130486163309, -287.9331878888522169, -229.8412257977494164 ) ) ;
#69155=CARTESIAN_POINT ( 'NONE',  ( -0.8642176097822394931, -276.5138609750960086, -204.4085972454281830 ) ) ;
#69156=CARTESIAN_POINT ( 'NONE',  ( -67.56613687916350841, -276.2348973475908451, -340.7492714063686208 ) ) ;
#69158=CARTESIAN_POINT ( 'NONE',  ( -36.17713848653617958, -297.2635566339611728, -193.5227470404294081 ) ) ;
#69159=CARTESIAN_POINT ( 'NONE',  ( 26.23471270372015596, -274.3058924017101958, -308.2558899628895688 ) ) ;
#69160=CARTESIAN_POINT ( 'NONE',  ( 1.165382885659398182, -278.6499945637035580, -206.5949340252136892 ) ) ;
#69161=CARTESIAN_POINT ( 'NONE',  ( -48.95330406819405766, -275.1061581843280806, -197.8369035123738513 ) ) ;
#69162=CARTESIAN_POINT ( 'NONE',  ( -1.858511850691574985, -274.9899250483807691, -337.7954101990465006 ) ) ;
#69164=CARTESIAN_POINT ( 'NONE',  ( -103.3006124605445564, -273.6292065093160772, -238.8442248656458275 ) ) ;
#69166=CARTESIAN_POINT ( 'NONE',  ( 13.47550346692731260, -286.3655769213731901, -326.0736839936324145 ) ) ;
#69167=CARTESIAN_POINT ( 'NONE',  ( 25.27692151142132104, -274.8681822947537512, -232.7410999281489694 ) ) ;
#69168=CARTESIAN_POINT ( 'NONE',  ( 39.64005161437589209, -287.5311880329594487, -268.6848427477963810 ) ) ;
#69169=CARTESIAN_POINT ( 'NONE',  ( -46.02760227429062923, -288.8260273098534867, -346.9014801462115543 ) ) ;
#69170=CARTESIAN_POINT ( 'NONE',  ( -35.89361067862525090, -300.0500808513247648, -195.0054237258406999 ) ) ;
#69171=CARTESIAN_POINT ( 'NONE',  ( -35.63367922416287570, -293.0305454694981790, -345.1877711499467978 ) ) ;
#69172=CARTESIAN_POINT ( 'NONE',  ( 36.44751926472988401, -280.4794686023626582, -248.8824091577034778 ) ) ;
#69173=DIRECTION ( 'NONE',  ( -1.000000000000000000, -0.000000000000000000, -0.000000000000000000 ) ) ;
#69174=CARTESIAN_POINT ( 'NONE',  ( -99.57556123191122310, -277.1183276717264903, -228.4820149166808676 ) ) ;
#69176=CARTESIAN_POINT ( 'NONE',  ( -87.00930905645846281, -288.5567837569653307, -324.4695016943931591 ) ) ;
#69179=CARTESIAN_POINT ( 'NONE',  ( -110.0410055481184060, -288.7894100584843500, -251.8749775035765026 ) ) ;
#69180=CARTESIAN_POINT ( 'NONE',  ( -3.806295163463269127, -276.0229930234823996, -204.7261916807048578 ) ) ;
#69181=CARTESIAN_POINT ( 'NONE',  ( 37.09930863393419997, -282.7595183661034071, -253.0658691171516068 ) ) ;
#69182=CARTESIAN_POINT ( 'NONE',  ( -108.7331577904153335, -270.9499913748800282, -245.6108862693309334 ) ) ;
#69183=CARTESIAN_POINT ( 'NONE',  ( -108.7200628095166763, -284.3495196044772797, -285.7217736511791486 ) ) ;
#69184=CARTESIAN_POINT ( 'NONE',  ( -64.80540891476478293, -275.1116061424378927, -202.0751348932619464 ) ) ;
#69185=CARTESIAN_POINT ( 'NONE',  ( -16.60466231704504025, -275.1297316148242658, -200.1472167058889227 ) ) ;
#69186=CARTESIAN_POINT ( 'NONE',  ( 8.019941878355446363, -284.4322384319294770, -330.0881811967416866 ) ) ;
#69187=CARTESIAN_POINT ( 'NONE',  ( -36.46788982174913940, -297.1221009679233021, -197.1259658601755973 ) ) ;
#69190=CARTESIAN_POINT ( 'NONE',  ( 13.39423242910156553, -294.1987229847631511, -328.3530086978565805 ) ) ;
#69191=CARTESIAN_POINT ( 'NONE',  ( -65.74186254280407127, -287.6588843635568651, -201.2750983082859761 ) ) ;
#69193=CARTESIAN_POINT ( 'NONE',  ( -55.56934967048407970, -277.3380690714490129, -190.3538533559490702 ) ) ;
#69194=CARTESIAN_POINT ( 'NONE',  ( -104.8386282014230630, -277.2731590543393736, -307.0806430435176253 ) ) ;
#69196=CARTESIAN_POINT ( 'NONE',  ( -101.6373126356855181, -288.4092470070361856, -311.3546454658352332 ) ) ;
#69197=CARTESIAN_POINT ( 'NONE',  ( -29.35040928699174501, -284.4693565499903798, -343.6708692461893975 ) ) ;
#69198=CARTESIAN_POINT ( 'NONE',  ( -104.0345266862015734, -279.8826139311257748, -302.5738828140925420 ) ) ;
#69199=CARTESIAN_POINT ( 'NONE',  ( -80.61953699863192924, -286.9034660038551579, -207.3239533732535733 ) ) ;
#69200=CARTESIAN_POINT ( 'NONE',  ( -8.501176363250989354, -282.4298136080363975, -201.1279984562739003 ) ) ;
#69201=CARTESIAN_POINT ( 'NONE',  ( -1.303373629501783704, -274.6834726146394701, -202.3152582429418942 ) ) ;
#69202=CARTESIAN_POINT ( 'NONE',  ( -72.84257142225602877, -277.3425458995909594, -338.7036210802558003 ) ) ;
#69203=CARTESIAN_POINT ( 'NONE',  ( -56.14386852559702135, -297.2162425734469480, -342.4408625498203378 ) ) ;
#69206=CARTESIAN_POINT ( 'NONE',  ( -40.36682480728010347, -296.1542282064546043, -194.6054403054197621 ) ) ;
#69207=CARTESIAN_POINT ( 'NONE',  ( 9.698888311416199670, -275.8916021848230002, -326.2643511692858738 ) ) ;
#69208=CARTESIAN_POINT ( 'NONE',  ( -80.46262503497078455, -298.5626496516304655, -206.8774031763040284 ) ) ;
#69209=CARTESIAN_POINT ( 'NONE',  ( 34.00013390127604396, -289.0554681077743453, -250.6553641942012121 ) ) ;
#69210=CARTESIAN_POINT ( 'NONE',  ( -112.4600240174401904, -298.2415588462148435, -256.9467536749043575 ) ) ;
#69211=CARTESIAN_POINT ( 'NONE',  ( -113.2569836957410843, -297.6236061545674829, -280.9900518570369741 ) ) ;
#69212=CARTESIAN_POINT ( 'NONE',  ( -78.27884800997664172, -293.5002010137922639, -207.7178553907379523 ) ) ;
#69213=CARTESIAN_POINT ( 'NONE',  ( -97.87405260181819244, -277.1527077894652393, -226.3626778668180464 ) ) ;
#69214=CARTESIAN_POINT ( 'NONE',  ( -110.5526814306512620, -280.6465741234623010, -256.8901708507413559 ) ) ;
#69215=CARTESIAN_POINT ( 'NONE',  ( -71.09913707219612888, -295.6829560375836650, -204.0012508289246398 ) ) ;
#69216=CARTESIAN_POINT ( 'NONE',  ( -67.36966247387626083, -285.3022068839415510, -339.9213577737837682 ) ) ;
#69217=CARTESIAN_POINT ( 'NONE',  ( 13.36324082226746413, -285.7018724636245111, -217.3454837400828126 ) ) ;
#69218=CARTESIAN_POINT ( 'NONE',  ( 123.2264321157264391, 148.5360561407864850, -263.2575006249301168 ) ) ;
#69220=CARTESIAN_POINT ( 'NONE',  ( 35.14469227722530320, -287.3351994146748893, -279.1821384915217550 ) ) ;
#69222=CARTESIAN_POINT ( 'NONE',  ( -1.765278710261730666, -283.6715999781039272, -338.3008762224394559 ) ) ;
#69223=CARTESIAN_POINT ( 'NONE',  ( -97.86309523353898498, -273.4542249049417819, -229.4144698171547816 ) ) ;
#69224=CARTESIAN_POINT ( 'NONE',  ( 23.55516425774165157, -285.7240790668212753, -223.8683178387225610 ) ) ;
#69225=CARTESIAN_POINT ( 'NONE',  ( -1.256671603243712410, -281.4602309328722072, -202.6064802828197742 ) ) ;
#69227=CARTESIAN_POINT ( 'NONE',  ( -19.93338039395358052, -281.7919569134650715, -196.0124422787080505 ) ) ;
#69228=CARTESIAN_POINT ( 'NONE',  ( -2.403531427808004661, -280.8348773736983617, -201.7528916542626121 ) ) ;
#69229=CARTESIAN_POINT ( 'NONE',  ( -82.08285599513421005, -282.9094976428776249, -214.2051214447836571 ) ) ;
#69230=CARTESIAN_POINT ( 'NONE',  ( 103.8745525416007496, 116.1007460503243607, -283.0288680581506355 ) ) ;
#69232=CARTESIAN_POINT ( 'NONE',  ( -54.65992989471284602, -275.8292287715964903, -197.5592818716456520 ) ) ;
#69233=CARTESIAN_POINT ( 'NONE',  ( -110.6039295111287544, -266.3419550533109259, -306.8688986251918323 ) ) ;
#69234=CARTESIAN_POINT ( 'NONE',  ( 28.28952166637291654, -280.0467606568328733, -305.9193733629799112 ) ) ;
#69235=CARTESIAN_POINT ( 'NONE',  ( 37.81759593152978027, -295.4540113672994721, -281.5438828316768536 ) ) ;
#69236=CARTESIAN_POINT ( 'NONE',  ( -26.20004334799273948, -294.2551394079507645, -342.6089978970040306 ) ) ;
#69237=CARTESIAN_POINT ( 'NONE',  ( -22.19975866122103980, -291.7486162255135582, -194.8730986231747124 ) ) ;
#69239=CARTESIAN_POINT ( 'NONE',  ( -92.28602029857157163, -294.3938677875706844, -323.4622288322950112 ) ) ;
#69240=CARTESIAN_POINT ( 'NONE',  ( 18.41671371781579580, -286.6342838432111648, -318.7846799880942399 ) ) ;
#69241=CARTESIAN_POINT ( 'NONE',  ( 35.15096508368568351, -295.2043822410277016, -254.3124578910395712 ) ) ;
#69242=CARTESIAN_POINT ( 'NONE',  ( 36.12217363706486850, -286.2820244621223083, -273.7994906670598994 ) ) ;
#69243=CARTESIAN_POINT ( 'NONE',  ( -95.35659980119862666, -286.4989386854391000, -225.2239969332456440 ) ) ;
#69245=CARTESIAN_POINT ( 'NONE',  ( 35.22624047049254870, -294.1750489317341248, -245.1660271171927548 ) ) ;
#69246=CARTESIAN_POINT ( 'NONE',  ( 32.29188160470507540, -282.3394509740934382, -292.6427317032751603 ) ) ;
#69247=CARTESIAN_POINT ( 'NONE',  ( -113.7235956879930399, -295.4284451834167839, -263.8886521477987799 ) ) ;
#69248=CARTESIAN_POINT ( 'NONE',  ( -113.0147736945237966, -291.5220680507783300, -257.0290229574998762 ) ) ;
#69249=CARTESIAN_POINT ( 'NONE',  ( -73.41041876034066149, -292.0791478858488972, -202.3861351202400272 ) ) ;
#69250=CARTESIAN_POINT ( 'NONE',  ( -10.72212113880805617, -288.8618850755676135, -338.3888442385951976 ) ) ;
#69253=CARTESIAN_POINT ( 'NONE',  ( -92.76940719763844356, -297.6967338247578141, -322.0336289705962258 ) ) ;
#69254=CARTESIAN_POINT ( 'NONE',  ( 52.88111462291031017, -297.8442732174480057, -193.8739110169187541 ) ) ;
#69255=CARTESIAN_POINT ( 'NONE',  ( 25.34387178002038610, -280.0901798291656633, -232.3955815017435782 ) ) ;
#69257=CARTESIAN_POINT ( 'NONE',  ( 30.48585073910440713, -275.5308438472565626, -306.7909476733175893 ) ) ;
#69258=CARTESIAN_POINT ( 'NONE',  ( -58.08154585589248597, -296.2591376933737592, -199.6464338632072781 ) ) ;
#69259=CARTESIAN_POINT ( 'NONE',  ( -29.56079077309719239, -278.8131378396576565, -344.2391887151030119 ) ) ;
#69260=CARTESIAN_POINT ( 'NONE',  ( 10.29556459549709224, -272.8566925253235809, -213.3591157503087459 ) ) ;
#69261=CARTESIAN_POINT ( 'NONE',  ( -58.50816103026473769, -296.5370856815455340, -340.6399301298143882 ) ) ;
#69262=CARTESIAN_POINT ( 'NONE',  ( -55.38298001842601792, -298.8943441392891600, -199.2541089461053332 ) ) ;
#69264=CARTESIAN_POINT ( 'NONE',  ( -108.6813058152199432, -297.8082822354275550, -297.2886207814248110 ) ) ;
#69265=CARTESIAN_POINT ( 'NONE',  ( -110.2208797385357286, -270.8196446865079565, -251.0035832070425386 ) ) ;
#69266=CARTESIAN_POINT ( 'NONE',  ( -38.90806881155080532, -292.6834012793393640, -197.2759679337297314 ) ) ;
#69267=CARTESIAN_POINT ( 'NONE',  ( -107.5584459396347370, -289.4169141798775513, -248.2963610346981227 ) ) ;
#69269=CARTESIAN_POINT ( 'NONE',  ( -21.37368610867320484, -274.7440150958080380, -195.0979169389452466 ) ) ;
#69270=CARTESIAN_POINT ( 'NONE',  ( -81.07270386167502352, -273.6062286352672004, -211.8460037010188728 ) ) ;
#69271=CARTESIAN_POINT ( 'NONE',  ( 24.90734321336867296, -282.9586211390911785, -227.8029091420009706 ) ) ;
#69272=CARTESIAN_POINT ( 'NONE',  ( -16.29369088238053465, -281.4705758751784401, -343.9706484194546192 ) ) ;
#69273=CARTESIAN_POINT ( 'NONE',  ( -17.39234758856538221, -276.1498424671655698, -344.6264269736359438 ) ) ;
#69274=CARTESIAN_POINT ( 'NONE',  ( -110.4704261979584032, -283.7781257015364531, -268.1722484470649874 ) ) ;
#69275=CARTESIAN_POINT ( 'NONE',  ( 1.133315503967222249, -280.5395511377577122, -334.9343446210174307 ) ) ;
#69276=CARTESIAN_POINT ( 'NONE',  ( 33.80727929939043719, -274.3730551417065726, -289.1546712620323092 ) ) ;
#69277=CARTESIAN_POINT ( 'NONE',  ( -93.76812529164524790, -281.2391512508279448, -220.8778602240109592 ) ) ;
#69280=CARTESIAN_POINT ( 'NONE',  ( -34.07830763726472867, -296.3323406979883998, -194.3754068573094003 ) ) ;
#69281=CARTESIAN_POINT ( 'NONE',  ( -105.8933992100000410, -280.1474408776773544, -301.3209834162412903 ) ) ;
#69283=CARTESIAN_POINT ( 'NONE',  ( -64.70742701758980786, -285.3268371164436985, -340.8053827262196478 ) ) ;
#69286=CARTESIAN_POINT ( 'NONE',  ( 25.19340208255916380, -286.1122329376198650, -311.8584847024332021 ) ) ;
#69288=CARTESIAN_POINT ( 'NONE',  ( -72.32728988598383069, -294.3208725906686709, -334.8978575460146772 ) ) ;
#69289=CARTESIAN_POINT ( 'NONE',  ( -64.29103499604589445, -287.5470180804531992, -339.5870223161121544 ) ) ;
#69291=CARTESIAN_POINT ( 'NONE',  ( -93.32116580629005398, -295.2467577490175472, -220.4481930762391642 ) ) ;
#69292=CARTESIAN_POINT ( 'NONE',  ( -75.74092574302582648, -284.0296335504341982, -204.3593413916691190 ) ) ;
#69293=CARTESIAN_POINT ( 'NONE',  ( -4.004221230905659290, -282.0994657437091178, -204.5059574697724543 ) ) ;
#69294=CARTESIAN_POINT ( 'NONE',  ( 33.38950778090992344, -279.4336669247442728, -242.4492455671945663 ) ) ;
#69295=CARTESIAN_POINT ( 'NONE',  ( -45.36244843969432594, -289.1566037294502394, -342.9191471490262302 ) ) ;
#69296=CARTESIAN_POINT ( 'NONE',  ( -68.79144662499599860, -281.0556376148206823, -203.8307612698487503 ) ) ;
#69297=CARTESIAN_POINT ( 'NONE',  ( -74.59680201176173853, -280.3459612062362680, -207.3373447454603138 ) ) ;
#69299=CARTESIAN_POINT ( 'NONE',  ( 35.55971737992850734, -289.7759980750545310, -289.4344011550113578 ) ) ;
#69301=CARTESIAN_POINT ( 'NONE',  ( -76.43272161342319748, -273.5448347711234192, -203.9602894325051921 ) ) ;
#69302=CARTESIAN_POINT ( 'NONE',  ( -95.36732255047787987, -291.8824715678344432, -317.3172033120404762 ) ) ;
#69304=CARTESIAN_POINT ( 'NONE',  ( 40.65961533371913106, -290.2662352645559167, -288.1317622949166548 ) ) ;
#69306=CARTESIAN_POINT ( 'NONE',  ( 11.49372615785818574, -274.3764101298928608, -327.5024302101932108 ) ) ;
#69308=CARTESIAN_POINT ( 'NONE',  ( -2.353145382731069546, -292.9968452683397118, -338.0533734794150291 ) ) ;
#69309=CARTESIAN_POINT ( 'NONE',  ( -95.33409194151947474, -296.6846996281569773, -225.9012151161579709 ) ) ;
#69310=CARTESIAN_POINT ( 'NONE',  ( -18.27563170611723820, -290.3222400462855717, -341.5984242092235377 ) ) ;
#69311=CARTESIAN_POINT ( 'NONE',  ( -83.40815489732948151, -285.4532926610873460, -328.3566151343581510 ) ) ;
#69312=CARTESIAN_POINT ( 'NONE',  ( -102.7211617983520000, -292.4987175454272119, -230.7099522497011606 ) ) ;
#69313=CARTESIAN_POINT ( 'NONE',  ( -61.54852897498791719, -293.0594195068215413, -197.7289585370036207 ) ) ;
#69314=CARTESIAN_POINT ( 'NONE',  ( -68.39850958073731135, -287.6443072045177587, -202.0934445279293925 ) ) ;
#69315=CARTESIAN_POINT ( 'NONE',  ( -84.56860703283433622, -279.5889427892554977, -209.4773675643675404 ) ) ;
#69316=CARTESIAN_POINT ( 'NONE',  ( -108.9882106666822068, -294.3240086637433137, -294.3630288440068057 ) ) ;
#69317=CARTESIAN_POINT ( 'NONE',  ( -66.57821600046094090, -283.2579563819441546, -341.6089067039796419 ) ) ;
#69318=CARTESIAN_POINT ( 'NONE',  ( -2.352044767130743175, -276.3807553175748808, -204.8890666943467807 ) ) ;
#69320=CARTESIAN_POINT ( 'NONE',  ( -92.05005921254146983, -280.4090924074130839, -314.0302885647153062 ) ) ;
#69321=CARTESIAN_POINT ( 'NONE',  ( -84.12262183171560537, -275.8266463380884375, -330.0252037396156766 ) ) ;
#69323=CARTESIAN_POINT ( 'NONE',  ( 17.64704285392907934, -281.7456241592662991, -318.4675269843156116 ) ) ;
#69324=CARTESIAN_POINT ( 'NONE',  ( -112.6723356732494921, -279.5815358763037466, -284.3364924590230203 ) ) ;
#69325=CARTESIAN_POINT ( 'NONE',  ( -33.72638223235642130, -285.1553578358346499, -193.6815920980390331 ) ) ;
#69326=CARTESIAN_POINT ( 'NONE',  ( -37.57534318073167867, -293.8093657382221409, -196.3355339494858924 ) ) ;
#69327=CARTESIAN_POINT ( 'NONE',  ( 37.42977496804506643, -276.9666831397738065, -255.6755151940899395 ) ) ;
#69328=CARTESIAN_POINT ( 'NONE',  ( 15.67317711600109043, -276.0990007206884229, -215.2002526639491293 ) ) ;
#69329=CARTESIAN_POINT ( 'NONE',  ( 32.89727594926724663, -275.6489238994626021, -290.2936939179304545 ) ) ;
#69330=CARTESIAN_POINT ( 'NONE',  ( -64.20388122450974322, -297.4034475819129852, -340.2619259435887216 ) ) ;
#69331=CARTESIAN_POINT ( 'NONE',  ( -112.2251689236907310, -282.5450820954114874, -270.8976449407572886 ) ) ;
#69332=CARTESIAN_POINT ( 'NONE',  ( -25.02064184023286231, -291.8719041091303552, -194.3746993663606588 ) ) ;
#69333=CARTESIAN_POINT ( 'NONE',  ( 38.55586450579806268, -289.0594273390983631, -263.0139173236334500 ) ) ;
#69334=CARTESIAN_POINT ( 'NONE',  ( 16.97643238134160626, -291.7693628098492127, -221.0548846136896373 ) ) ;
#69336=CARTESIAN_POINT ( 'NONE',  ( 30.38513866485025261, -291.6656358304941818, -234.8680488545314518 ) ) ;
#69337=CARTESIAN_POINT ( 'NONE',  ( -67.80614379073990960, -291.3076832542452053, -203.9847011862297563 ) ) ;
#69339=CARTESIAN_POINT ( 'NONE',  ( -59.92308945573012835, -290.4177618427382868, -343.6521362938286757 ) ) ;
#69340=CARTESIAN_POINT ( 'NONE',  ( -109.6433618957493366, -279.0249137139012419, -259.7848067016466871 ) ) ;
#69341=CARTESIAN_POINT ( 'NONE',  ( -102.8586806540441074, -294.9498851330534421, -310.2236037553919914 ) ) ;
#69342=CARTESIAN_POINT ( 'NONE',  ( -93.85047565060217778, -285.9152642450737289, -218.1287687468918080 ) ) ;
#69343=CARTESIAN_POINT ( 'NONE',  ( 12.06075724195058285, -287.0504729443960059, -211.2564775508933508 ) ) ;
#69345=CARTESIAN_POINT ( 'NONE',  ( -108.9505344823494539, -285.0739155887426932, -256.0690807143886900 ) ) ;
#69346=CARTESIAN_POINT ( 'NONE',  ( -84.39908107231754286, -219.2962774960428760, -352.3863144506401568 ) ) ;
#69347=CARTESIAN_POINT ( 'NONE',  ( -49.37733225207519183, -154.2223004629079810, -363.8550686714801827 ) ) ;
#69348=CARTESIAN_POINT ( 'NONE',  ( -83.36829938135619500, -218.4018712402734650, -348.9267425600256161 ) ) ;
#69349=CARTESIAN_POINT ( 'NONE',  ( 35.18192278478999668, -274.6224313375963675, -260.7213126656877193 ) ) ;
#69350=CARTESIAN_POINT ( 'NONE',  ( 31.54753624136908030, -274.8068624756293730, -295.5784400796692921 ) ) ;
#69351=CARTESIAN_POINT ( 'NONE',  ( -68.14705418104928469, -297.1661347181519659, -199.8021905112523484 ) ) ;
#69352=CARTESIAN_POINT ( 'NONE',  ( -11.27636105762056218, -93.00928234723599530, -356.9605620023007759 ) ) ;
#69353=CARTESIAN_POINT ( 'NONE',  ( 24.93528355352991355, -273.6443032015265544, -225.8991278562868104 ) ) ;
#69354=CARTESIAN_POINT ( 'NONE',  ( -89.97836760152866020, -275.0560971070458436, -218.3288659641350193 ) ) ;
#69355=CARTESIAN_POINT ( 'NONE',  ( 53.23043170612119468, -300.1013752903952536, -193.5822955068719580 ) ) ;
#69356=CARTESIAN_POINT ( 'NONE',  ( 33.14294324827755389, -288.3006089749009675, -289.7817941462497515 ) ) ;
#69357=CARTESIAN_POINT ( 'NONE',  ( -47.59987637687407158, -295.9822399706359874, -346.5118148947088343 ) ) ;
#69358=CARTESIAN_POINT ( 'NONE',  ( -43.29125860421211058, -298.4714041380003664, -193.5998693973546665 ) ) ;
#69359=CARTESIAN_POINT ( 'NONE',  ( -36.99341668510393788, -295.2143193158671579, -343.3727113808294007 ) ) ;
#69361=CARTESIAN_POINT ( 'NONE',  ( 12.98676805008828516, -276.6682520112348698, -213.9320191820249306 ) ) ;
#69363=CARTESIAN_POINT ( 'NONE',  ( -62.02194941492411573, -279.2474761315834257, -197.4323570711135574 ) ) ;
#69365=CARTESIAN_POINT ( 'NONE',  ( -59.25401880934609977, -278.2841331671683065, -340.2414352233124646 ) ) ;
#69366=CARTESIAN_POINT ( 'NONE',  ( 16.25656700619970607, -278.0645506452200379, -324.2974006643162852 ) ) ;
#69367=CARTESIAN_POINT ( 'NONE',  ( -112.5673809534716412, -276.6286952785854965, -265.9448135772202590 ) ) ;
#69368=CARTESIAN_POINT ( 'NONE',  ( -31.34090078994525186, -274.6222994094842988, -197.5337693306901201 ) ) ;
#69369=CARTESIAN_POINT ( 'NONE',  ( -95.24824955063338905, -294.4916823707704907, -315.7726413329684760 ) ) ;
#69371=CARTESIAN_POINT ( 'NONE',  ( -92.72525199358497616, -278.0417474314594983, -317.9180542514714034 ) ) ;
#69372=CARTESIAN_POINT ( 'NONE',  ( 20.19092575943044565, -286.9238835169735466, -320.8119428413362471 ) ) ;
#69373=CARTESIAN_POINT ( 'NONE',  ( -91.73956980718394050, -275.2768696529319072, -218.7102821747882331 ) ) ;
#69375=CARTESIAN_POINT ( 'NONE',  ( -109.7842798137740061, -289.6134650260669900, -280.6821334575872129 ) ) ;
#69376=CARTESIAN_POINT ( 'NONE',  ( -93.36297077219080620, -283.1806396571025175, -323.0580291428240685 ) ) ;
#69377=CARTESIAN_POINT ( 'NONE',  ( 34.29878201119488068, -280.0346712132531479, -289.0022723677582803 ) ) ;
#69378=CARTESIAN_POINT ( 'NONE',  ( 36.27727800054010743, -280.1036604844420594, -268.5873393084081613 ) ) ;
#69379=CARTESIAN_POINT ( 'NONE',  ( -110.8390699916720337, -282.7858038708150161, -258.4716102760308445 ) ) ;
#69380=CARTESIAN_POINT ( 'NONE',  ( -101.0618137784083927, -287.0846222468462656, -230.7079353797111025 ) ) ;
#69381=CARTESIAN_POINT ( 'NONE',  ( -108.0047395983793024, -280.0186916642916231, -250.4684590381736768 ) ) ;
#69383=CARTESIAN_POINT ( 'NONE',  ( -41.95701226949705642, -293.9941322649137305, -195.5032557114952851 ) ) ;
#69384=CARTESIAN_POINT ( 'NONE',  ( -79.68042081936802390, -275.8552945232693787, -333.5228601610585315 ) ) ;
#69385=CARTESIAN_POINT ( 'NONE',  ( -29.69452379241713658, -277.6043300044238435, -343.1129437645186613 ) ) ;
#69386=CARTESIAN_POINT ( 'NONE',  ( -108.4811609076313772, -286.2390008513100952, -294.6346744947704792 ) ) ;
#69387=FACE_OUTER_BOUND ( 'NONE', #13266, .T. ) ;
#69388=CARTESIAN_POINT ( 'NONE',  ( -94.35537848841242692, -291.7892380602669391, -319.9469494255017139 ) ) ;
#69389=CARTESIAN_POINT ( 'NONE',  ( -63.94642986785227379, -293.3988062045393690, -340.5384513318622908 ) ) ;
#69390=CARTESIAN_POINT ( 'NONE',  ( 39.44242436935382301, -286.8002474509322610, -274.4246113523318513 ) ) ;
#69391=CARTESIAN_POINT ( 'NONE',  ( -63.06063917047178791, -290.1114013042531496, -201.1875927756718738 ) ) ;
#69393=CARTESIAN_POINT ( 'NONE',  ( 15.94398068009744307, -274.9617416160315884, -320.9761325423675657 ) ) ;
#69394=CARTESIAN_POINT ( 'NONE',  ( -8.777125805074488696, -292.8140207091449270, -338.8945153180375200 ) ) ;
#69397=CARTESIAN_POINT ( 'NONE',  ( -92.29917155378441862, -289.7640534626253839, -217.3484180542841955 ) ) ;
#69398=CARTESIAN_POINT ( 'NONE',  ( -108.8084139374457351, -286.3926812883466368, -251.9505440025732241 ) ) ;
#69399=CARTESIAN_POINT ( 'NONE',  ( 30.76904521955583149, -286.2320741222289371, -304.1679973948490669 ) ) ;
#69400=CARTESIAN_POINT ( 'NONE',  ( -108.6037636650999048, -286.2178534755499300, -252.0010194256967964 ) ) ;
#69401=CARTESIAN_POINT ( 'NONE',  ( 121.3395553409046670, -299.5541904835127980, -198.1000099699160444 ) ) ;
#69402=CARTESIAN_POINT ( 'NONE',  ( -91.64793505991495692, -286.0562151238987099, -221.2618291277825904 ) ) ;
#69404=CARTESIAN_POINT ( 'NONE',  ( 31.91506390335319310, -295.9200497360366171, -300.1899273375339021 ) ) ;
#69406=CARTESIAN_POINT ( 'NONE',  ( -42.72837979928182506, -275.1994756122139734, -345.7288689153223231 ) ) ;
#69407=CARTESIAN_POINT ( 'NONE',  ( -9.215591531353517496, -277.0275857541622031, -342.0177039096741964 ) ) ;
#69408=CARTESIAN_POINT ( 'NONE',  ( -11.62001420522589257, -290.4642371877069422, -199.2588891646350362 ) ) ;
#69409=CARTESIAN_POINT ( 'NONE',  ( -114.0791115065781725, -278.4649831994051965, -277.3310780118933394 ) ) ;
#69410=CARTESIAN_POINT ( 'NONE',  ( -94.32199081411876307, -297.8616100733190137, -318.6001317323788271 ) ) ;
#69413=CARTESIAN_POINT ( 'NONE',  ( -52.17219592184963517, -284.5431086975402195, -198.3798713199116435 ) ) ;
#69414=CARTESIAN_POINT ( 'NONE',  ( -85.93132192577222384, -275.8729011566883855, -326.5533265629862854 ) ) ;
#69415=CARTESIAN_POINT ( 'NONE',  ( 24.27236515191030009, -280.1322721924374264, -313.1470853277362494 ) ) ;
#69417=CARTESIAN_POINT ( 'NONE',  ( 31.93183840629263415, -273.6175164064592877, -238.2370238571341474 ) ) ;
#69418=CARTESIAN_POINT ( 'NONE',  ( -99.26584843626726240, -277.3638847558975158, -309.3053025640978149 ) ) ;
#69419=CARTESIAN_POINT ( 'NONE',  ( 36.31369746165925250, -295.0413854402277707, -267.9967668029023002 ) ) ;
#69420=CARTESIAN_POINT ( 'NONE',  ( -5.061536280651216302, -279.3875655840416812, -200.7947214030889427 ) ) ;
#69421=CARTESIAN_POINT ( 'NONE',  ( 1.705393863920346975, -295.4575749099768132, -332.3786931559660047 ) ) ;
#69422=CARTESIAN_POINT ( 'NONE',  ( -100.3540685539231134, -298.4440960540918013, -226.9475399014949346 ) ) ;
#69423=CARTESIAN_POINT ( 'NONE',  ( -63.07747839314306759, -297.5408842529122921, -201.9946117079880139 ) ) ;
#69424=CARTESIAN_POINT ( 'NONE',  ( -98.40413833343902184, -293.1454919977227291, -226.7257971800193275 ) ) ;
#69425=CARTESIAN_POINT ( 'NONE',  ( -33.72945163228306598, -286.2631108636859949, -193.4458940972773746 ) ) ;
#69426=CARTESIAN_POINT ( 'NONE',  ( 35.68857311150232903, -273.9491126216996690, -290.5808188123639297 ) ) ;
#69427=CARTESIAN_POINT ( 'NONE',  ( -23.31402084651426421, -288.7110001825039944, -346.1266860558930603 ) ) ;
#69428=CARTESIAN_POINT ( 'NONE',  ( -103.6278531975442689, -280.9898281879271735, -235.9266545479738966 ) ) ;
#69430=CARTESIAN_POINT ( 'NONE',  ( 34.51269112357425684, -286.7978729038478036, -284.5805697825753100 ) ) ;
#69431=CARTESIAN_POINT ( 'NONE',  ( -80.75151250047828455, -289.4629772906923790, -209.2007645179615736 ) ) ;
#69433=CARTESIAN_POINT ( 'NONE',  ( -102.0362518552990423, -259.7623939308359695, -328.6249738900723969 ) ) ;
#69434=CARTESIAN_POINT ( 'NONE',  ( -61.28108940861380205, -288.8792550081258810, -339.3893302039106175 ) ) ;
#69436=CARTESIAN_POINT ( 'NONE',  ( -76.62714499559241688, -284.5052501248687236, -336.3732853822853031 ) ) ;
#69437=CARTESIAN_POINT ( 'NONE',  ( -40.61036776083165023, -291.0707700265456310, -193.6528912313968078 ) ) ;
#69438=CARTESIAN_POINT ( 'NONE',  ( 28.58414392714239582, -282.6501001470448955, -232.1482471207737035 ) ) ;
#69439=CARTESIAN_POINT ( 'NONE',  ( 39.14689015336591638, -282.8257966658646865, -267.0618306769619039 ) ) ;
#69440=CARTESIAN_POINT ( 'NONE',  ( 32.95887426622155658, -281.6454265011823281, -290.0290930778809297 ) ) ;
#69441=CARTESIAN_POINT ( 'NONE',  ( 23.89960802109775528, -276.9638032042099098, -227.0433675002260827 ) ) ;
#69442=CARTESIAN_POINT ( 'NONE',  ( -98.27445923397482375, -295.9237694725378560, -317.4376393891290604 ) ) ;
#69443=CARTESIAN_POINT ( 'NONE',  ( -96.26414359644908814, -287.9406642249805373, -316.2074531922903589 ) ) ;
#69444=CARTESIAN_POINT ( 'NONE',  ( -39.16228013766123439, -296.9491326165413057, -197.0621530590104840 ) ) ;
#69447=CARTESIAN_POINT ( 'NONE',  ( -111.8311986425008655, -286.4647658536589461, -270.9445170679634316 ) ) ;
#69448=CARTESIAN_POINT ( 'NONE',  ( 19.31066272960425323, -295.3380893840782164, -322.1298996623218045 ) ) ;
#69449=CARTESIAN_POINT ( 'NONE',  ( -65.34708510383936186, -284.0795494377312025, -337.8994789742364446 ) ) ;
#69450=CARTESIAN_POINT ( 'NONE',  ( -11.95534101051359954, -275.7885212533428216, -342.8623874599227292 ) ) ;
#69451=CARTESIAN_POINT ( 'NONE',  ( -99.12764888475417990, -291.8131947163757332, -224.5590464796171375 ) ) ;
#69452=CARTESIAN_POINT ( 'NONE',  ( -99.96200840901717299, -283.2644397458983008, -227.6187168763532327 ) ) ;
#69453=CARTESIAN_POINT ( 'NONE',  ( 11.10218649761893062, -293.0349503802119102, -210.4683474772775185 ) ) ;
#69454=CARTESIAN_POINT ( 'NONE',  ( -104.0653111308672720, -290.4846908128180303, -300.1515639711514609 ) ) ;
#69457=CARTESIAN_POINT ( 'NONE',  ( 196.8450047754690786, 281.6590421831631375, -110.2675066226584306 ) ) ;
#69458=CARTESIAN_POINT ( 'NONE',  ( -85.64836685764284141, -285.2269756160812335, -329.4303460151899117 ) ) ;
#69459=CARTESIAN_POINT ( 'NONE',  ( -106.6662871844225293, -281.6237833571634610, -303.7098442033569086 ) ) ;
#69461=CARTESIAN_POINT ( 'NONE',  ( 34.23927659396760248, -280.6803394542382080, -286.1848295005096929 ) ) ;
#69462=CARTESIAN_POINT ( 'NONE',  ( 10.50959377909168957, -276.0788510585550739, -330.7284183860144822 ) ) ;
#69463=CARTESIAN_POINT ( 'NONE',  ( -93.60320318817002772, -281.2394580563473028, -220.9992240685792240 ) ) ;
#69464=CARTESIAN_POINT ( 'NONE',  ( 191.1870090034608722, 268.7882272122546965, -138.6016306282632229 ) ) ;
#69465=CARTESIAN_POINT ( 'NONE',  ( 12.62070560280848319, -279.3077516454175111, -212.5479334572429764 ) ) ;
#69466=CARTESIAN_POINT ( 'NONE',  ( -110.5369872706778125, -282.7611163219394825, -255.7222400936766746 ) ) ;
#69467=CARTESIAN_POINT ( 'NONE',  ( -35.87538550795238734, -299.8304042988154947, -194.3740123294689965 ) ) ;
#69468=CARTESIAN_POINT ( 'NONE',  ( -108.0275227610104167, -296.8001298739014260, -288.8903634243297915 ) ) ;
#69470=CARTESIAN_POINT ( 'NONE',  ( -101.5464035355524288, -289.7239590354090524, -234.4935303490441356 ) ) ;
#69471=CARTESIAN_POINT ( 'NONE',  ( -25.77710018954696025, -277.5599348301415716, -346.3846197080057436 ) ) ;
#69472=CARTESIAN_POINT ( 'NONE',  ( -27.29017932440858019, -274.1833156033798673, -198.0055382361872205 ) ) ;
#69473=CARTESIAN_POINT ( 'NONE',  ( 28.82229840856515324, -274.9792990288836450, -309.1402077959008921 ) ) ;
#69475=CARTESIAN_POINT ( 'NONE',  ( -109.1535629427707761, -270.8328122144964709, -248.5502976032099696 ) ) ;
#69479=CARTESIAN_POINT ( 'NONE',  ( -38.87782810695519942, -284.1515094091836886, -343.6666792295779373 ) ) ;
#69480=CARTESIAN_POINT ( 'NONE',  ( -8.403753812197678030, -284.4387593180005638, -340.6776451799821643 ) ) ;
#69482=CARTESIAN_POINT ( 'NONE',  ( -107.4503514271510767, -284.1764063920904846, -249.4812855012324064 ) ) ;
#69483=CARTESIAN_POINT ( 'NONE',  ( 8.056652841658774378, -274.8199126588855847, -328.6106691162278253 ) ) ;
#69484=CARTESIAN_POINT ( 'NONE',  ( 8.576272517067319967, -284.2763221306306605, -328.7569247596914579 ) ) ;
#69485=CARTESIAN_POINT ( 'NONE',  ( -93.26530470542337525, -276.3552181164891408, -318.3533903285371593 ) ) ;
#69486=CARTESIAN_POINT ( 'NONE',  ( 114.7448031289451222, -299.5541904835127980, -198.3007743052732792 ) ) ;
#69488=CARTESIAN_POINT ( 'NONE',  ( -111.9316427951227411, -279.5869213807203550, -251.8544833326130004 ) ) ;
#69492=CARTESIAN_POINT ( 'NONE',  ( -101.4855418731528403, -286.9491505258046686, -230.0390018973986628 ) ) ;
#69494=CARTESIAN_POINT ( 'NONE',  ( 1.647256885009238392, -293.7137714050210775, -332.3280024614030594 ) ) ;
#69495=CARTESIAN_POINT ( 'NONE',  ( -93.52400366868117487, -289.1831090167933098, -322.9436931885342119 ) ) ;
#69496=CARTESIAN_POINT ( 'NONE',  ( 13.85648495682666770, -285.0215122446341525, -216.8420967159271129 ) ) ;
#69497=CARTESIAN_POINT ( 'NONE',  ( 19.12547874439903950, -285.4622756829367063, -223.1521526243907658 ) ) ;
#69498=CARTESIAN_POINT ( 'NONE',  ( -105.6294734056318845, -289.1712406661733326, -241.6839482297548329 ) ) ;
#69499=CARTESIAN_POINT ( 'NONE',  ( -109.8156424661205222, -285.9105290961912260, -258.6771736978408853 ) ) ;
#69500=CARTESIAN_POINT ( 'NONE',  ( 30.04677536129861082, -273.9873451767913934, -303.4003539869329416 ) ) ;
#69501=CARTESIAN_POINT ( 'NONE',  ( 29.44036529408687386, -285.4705646659645595, -233.5555854469791939 ) ) ;
#69502=CARTESIAN_POINT ( 'NONE',  ( -99.11814275560450938, -299.1289719495663348, -227.8100562063340817 ) ) ;
#69503=CARTESIAN_POINT ( 'NONE',  ( 23.24112150529521870, -284.9465970999091837, -225.8667346073227122 ) ) ;
#69504=CARTESIAN_POINT ( 'NONE',  ( -7.915870426184912212, -281.3886525869224897, -203.2837836643297749 ) ) ;
#69505=CARTESIAN_POINT ( 'NONE',  ( -34.70500001451793537, -291.0192456441765216, -345.4815296015473223 ) ) ;
#69508=CARTESIAN_POINT ( 'NONE',  ( -85.45914795579160739, -297.6316861945697383, -328.6193827157596274 ) ) ;
#69509=CARTESIAN_POINT ( 'NONE',  ( -101.1564221430063242, -277.0820326420379160, -230.8580107957405403 ) ) ;
#69510=CARTESIAN_POINT ( 'NONE',  ( -30.70101279077371004, -291.3311158970092265, -193.7574409809942324 ) ) ;
#69511=CARTESIAN_POINT ( 'NONE',  ( -80.17599929689119165, -295.8611025512300898, -210.2640030096187616 ) ) ;
#69512=CARTESIAN_POINT ( 'NONE',  ( 17.96500432436192796, -280.9229303009006458, -318.7595882219055738 ) ) ;
#69513=CARTESIAN_POINT ( 'NONE',  ( -38.07243738793426502, -272.1227723196129773, -195.9247006543479301 ) ) ;
#69514=CARTESIAN_POINT ( 'NONE',  ( 18.84284627870105311, -294.1987148133409278, -222.9845391241362904 ) ) ;
#69515=CARTESIAN_POINT ( 'NONE',  ( 10.64812456238589888, -296.9090924074130271, -330.4860931364851808 ) ) ;
#69516=CARTESIAN_POINT ( 'NONE',  ( -108.7951894671945041, -294.6885344560242288, -297.2891440076819549 ) ) ;
#69517=CARTESIAN_POINT ( 'NONE',  ( 6.017152072562857335, -292.7131223114755585, -332.8270126763905523 ) ) ;
#69518=CARTESIAN_POINT ( 'NONE',  ( -98.59111584620231383, -291.4154237662127684, -311.1747844643946905 ) ) ;
#69520=CARTESIAN_POINT ( 'NONE',  ( -94.42330362243954767, -292.0005106644792932, -224.5777691534463258 ) ) ;
#69523=CARTESIAN_POINT ( 'NONE',  ( -1.187225902346443318, -280.5950860486489660, -336.4912467594318173 ) ) ;
#69524=CARTESIAN_POINT ( 'NONE',  ( 33.11670124815748295, -293.8049571239789088, -289.5035058035148268 ) ) ;
#69525=CARTESIAN_POINT ( 'NONE',  ( 27.85135275202823735, -281.0145239857965862, -229.2872291557859512 ) ) ;
#69526=CARTESIAN_POINT ( 'NONE',  ( -114.3196013377307025, -284.2236682712230618, -269.9776902938024250 ) ) ;
#69527=CARTESIAN_POINT ( 'NONE',  ( -48.35535419701226800, -287.1923465995993183, -344.4318521171526868 ) ) ;
#69528=CARTESIAN_POINT ( 'NONE',  ( -108.9589582432861903, -282.4373116804489996, -289.9497373114602397 ) ) ;
#69529=CARTESIAN_POINT ( 'NONE',  ( -31.11089127851601788, -278.6092638056593955, -194.2570459774840970 ) ) ;
#69530=CARTESIAN_POINT ( 'NONE',  ( -37.96607899856367396, -284.9648356159121931, -193.6727703522207662 ) ) ;
#69532=CARTESIAN_POINT ( 'NONE',  ( 30.23063850712377487, -295.5471272745234046, -300.0329811615882249 ) ) ;
#69533=CARTESIAN_POINT ( 'NONE',  ( -28.64989671812455896, -278.3693854571712905, -346.3290974306423209 ) ) ;
#69534=CARTESIAN_POINT ( 'NONE',  ( -110.1794365029900860, -278.2870790740148550, -265.1889185968924494 ) ) ;
#69535=CARTESIAN_POINT ( 'NONE',  ( -112.3177557784249530, -290.9381777740092048, -252.8228431628078283 ) ) ;
#69536=CARTESIAN_POINT ( 'NONE',  ( -19.28663378117657601, -280.9016039972770500, -343.7862150809997956 ) ) ;
#69537=CARTESIAN_POINT ( 'NONE',  ( 31.75808359013602455, -292.9344627656906823, -294.7745538413889790 ) ) ;
#69539=CARTESIAN_POINT ( 'NONE',  ( -110.3645422528903737, -294.3316239379112744, -287.5242054714675533 ) ) ;
#69542=CARTESIAN_POINT ( 'NONE',  ( -34.30490732508198448, -294.5205949036196671, -343.3595174942433914 ) ) ;
#69545=CARTESIAN_POINT ( 'NONE',  ( -105.5937364680635966, -293.8380690714490129, -285.9065529553535612 ) ) ;
#69546=CARTESIAN_POINT ( 'NONE',  ( -70.61617690632397171, -296.6827749010979005, -201.1828742247705293 ) ) ;
#69547=CARTESIAN_POINT ( 'NONE',  ( 25.27339112443712565, -279.1189327153433624, -227.6121128796392838 ) ) ;
#69548=CARTESIAN_POINT ( 'NONE',  ( -49.28437614253680010, -287.2182936830355402, -194.7387449098748391 ) ) ;
#69549=CARTESIAN_POINT ( 'NONE',  ( 32.31297602119136769, -287.6770031641011656, -292.3748472534764460 ) ) ;
#69550=CARTESIAN_POINT ( 'NONE',  ( -26.90436270166161137, -278.4371500327605986, -343.3115788357914084 ) ) ;
#69551=CARTESIAN_POINT ( 'NONE',  ( -107.5424911924934008, -294.2399679148196014, -295.8844054648898236 ) ) ;
#69552=CARTESIAN_POINT ( 'NONE',  ( -110.2782175177796660, -298.4759665512610809, -257.7818316049368832 ) ) ;
#69554=CARTESIAN_POINT ( 'NONE',  ( -103.4955181729308720, -276.9178740636837688, -302.2718954800412803 ) ) ;
#69556=CARTESIAN_POINT ( 'NONE',  ( -36.53663737784922461, -297.7286944007803413, -193.3823058181700105 ) ) ;
#69557=CARTESIAN_POINT ( 'NONE',  ( -96.90614746118225753, -291.8574368116718460, -315.0297871423659899 ) ) ;
#69558=CARTESIAN_POINT ( 'NONE',  ( 33.70942227791663726, -294.7981239755835077, -242.6803627348150201 ) ) ;
#69559=CARTESIAN_POINT ( 'NONE',  ( -113.5925053212108367, -274.1217662500657752, -270.3811029296526272 ) ) ;
#69561=CARTESIAN_POINT ( 'NONE',  ( -106.1256812250172317, -290.8743708587069818, -295.1130191723560756 ) ) ;
#69564=CARTESIAN_POINT ( 'NONE',  ( -107.6831522978168181, -297.6019857336125938, -239.1586606603594021 ) ) ;
#69565=CARTESIAN_POINT ( 'NONE',  ( -111.4270734077455387, -288.8941166746070053, -254.4361121468469662 ) ) ;
#69566=CARTESIAN_POINT ( 'NONE',  ( -48.97098675466904893, -298.2412898071205518, -194.2121049031047733 ) ) ;
#69569=CARTESIAN_POINT ( 'NONE',  ( -4.612731704203378413, -290.1489117453890003, -339.3067565660630294 ) ) ;
#69570=CARTESIAN_POINT ( 'NONE',  ( -2.659677404128715672, -276.9805209788415823, -198.2697987213421698 ) ) ;
#69571=CARTESIAN_POINT ( 'NONE',  ( -75.68071226403637297, -287.5393609505711083, -206.0948859875217920 ) ) ;
#69572=CARTESIAN_POINT ( 'NONE',  ( -10.18625753643228471, -284.9743684092888429, -198.8821429856936902 ) ) ;
#69573=CARTESIAN_POINT ( 'NONE',  ( -29.77990311428824199, -272.1479549997527556, -195.9108147473772306 ) ) ;
#69574=CARTESIAN_POINT ( 'NONE',  ( -32.62371850801106632, -276.0322066089227633, -196.0580029286489321 ) ) ;
#69575=CARTESIAN_POINT ( 'NONE',  ( -110.1132355926697670, -288.8347416479156777, -254.6889187880003647 ) ) ;
#69576=CARTESIAN_POINT ( 'NONE',  ( -31.52113279118070466, -278.8399530403050903, -345.9537895888056482 ) ) ;
#69579=CARTESIAN_POINT ( 'NONE',  ( -16.92171599363927825, -280.3233262224409259, -200.2752831230883714 ) ) ;
#69580=CARTESIAN_POINT ( 'NONE',  ( 34.80282127787744173, -281.0560806271518572, -282.1535180532416121 ) ) ;
#69581=CARTESIAN_POINT ( 'NONE',  ( 12.51413602631390809, -277.4557462844888960, -328.6353671004637249 ) ) ;
#69582=CARTESIAN_POINT ( 'NONE',  ( 36.94993633285494639, -280.1122101018423223, -251.6859614396394420 ) ) ;
#69583=CARTESIAN_POINT ( 'NONE',  ( 183.2096664736218941, 262.1940599670854226, -151.6038608880942604 ) ) ;
#69584=CARTESIAN_POINT ( 'NONE',  ( 22.46525358159449937, -277.1405311111119545, -318.5062170397638965 ) ) ;
#69585=CARTESIAN_POINT ( 'NONE',  ( 18.83135759094050599, -300.1677098511511872, -193.9370241457030772 ) ) ;
#69586=CARTESIAN_POINT ( 'NONE',  ( -69.91165696735023971, -294.1233781216987495, -202.8022627189028810 ) ) ;
#69589=CARTESIAN_POINT ( 'NONE',  ( 10.32664862597122202, -289.4561147116154984, -326.1234433550667973 ) ) ;
#69590=CARTESIAN_POINT ( 'NONE',  ( 37.02706177743279170, -289.1138289212092332, -254.7013684694493065 ) ) ;
#69591=CARTESIAN_POINT ( 'NONE',  ( -94.18878076761573936, -289.2515921764393170, -316.3209057467874459 ) ) ;
#69592=CARTESIAN_POINT ( 'NONE',  ( 16.26081180745041621, -286.2964823327575914, -215.1678428729391328 ) ) ;
#69593=CARTESIAN_POINT ( 'NONE',  ( 46.30223402071163008, 11.84457614133316739, -331.9951998377467248 ) ) ;
#69594=CARTESIAN_POINT ( 'NONE',  ( 34.09278559577506229, -280.1946581799574574, -288.9466275635909938 ) ) ;
#69595=CARTESIAN_POINT ( 'NONE',  ( -12.85852211518442978, -290.5909469464642712, -340.4427808746546589 ) ) ;
#69596=CARTESIAN_POINT ( 'NONE',  ( 16.31754883453841742, -280.7530912225772681, -320.9460301366980275 ) ) ;
#69597=CARTESIAN_POINT ( 'NONE',  ( -54.62490118411572126, -281.1406908207898141, -198.8765383312015729 ) ) ;
#69598=CARTESIAN_POINT ( 'NONE',  ( -87.13289349890753499, -278.2610595509717655, -323.8291037706811721 ) ) ;
#69599=CARTESIAN_POINT ( 'NONE',  ( -112.4815312297281480, -289.1589320936956824, -285.3278223799621287 ) ) ;
#69600=CARTESIAN_POINT ( 'NONE',  ( -80.85519803970743169, -286.2811265091950190, -206.9665304403151254 ) ) ;
#69601=CARTESIAN_POINT ( 'NONE',  ( -113.8420065473951439, -284.9418712398101547, -278.5605094777939144 ) ) ;
#69602=CARTESIAN_POINT ( 'NONE',  ( -13.52736033071201227, -282.9009932185252865, -339.4210794726359381 ) ) ;
#69605=CARTESIAN_POINT ( 'NONE',  ( -111.0553320826483628, -292.1892972883025550, -287.9267245971706188 ) ) ;
#69606=CARTESIAN_POINT ( 'NONE',  ( 23.59268187554334517, -291.6162989534926737, -224.0761843295774725 ) ) ;
#69607=CARTESIAN_POINT ( 'NONE',  ( -21.87267913420982879, -273.3140358340575062, -198.7781742259252553 ) ) ;
#69608=CARTESIAN_POINT ( 'NONE',  ( -107.0774262175834508, -295.4854319956171480, -302.7685444931653365 ) ) ;
#69610=CARTESIAN_POINT ( 'NONE',  ( -94.81962833724782058, -289.6779324196597258, -224.2217100824878173 ) ) ;
#69611=CARTESIAN_POINT ( 'NONE',  ( -45.22058505916535864, -293.3930169018261154, -344.0050752340478653 ) ) ;
#69612=CARTESIAN_POINT ( 'NONE',  ( -34.54759563645244214, -290.2214813549700807, -343.7548400750943642 ) ) ;
#69613=DIRECTION ( 'NONE',  ( 0.000000000000000000, 0.000000000000000000, -1.000000000000000000 ) ) ;
#69614=CARTESIAN_POINT ( 'NONE',  ( -96.56424898580104355, -291.9213121697696351, -316.3794877895917352 ) ) ;
#69615=CARTESIAN_POINT ( 'NONE',  ( 37.67065740580651578, -291.6233253230812466, -275.9293257105272232 ) ) ;
#69617=CARTESIAN_POINT ( 'NONE',  ( -17.64850385707197233, -296.7984314159474479, -342.7827073950271028 ) ) ;
#69618=CARTESIAN_POINT ( 'NONE',  ( 4.851173008370035511, -287.5787675610760061, -210.4394824881779584 ) ) ;
#69619=CARTESIAN_POINT ( 'NONE',  ( -6.525455917431348674, -296.6485726010029680, -338.9204902271051196 ) ) ;
#69620=CARTESIAN_POINT ( 'NONE',  ( 6.262250606421436494, -276.6203681421435476, -208.8389617503153488 ) ) ;
#69621=CARTESIAN_POINT ( 'NONE',  ( 18.60268395288361987, -275.0645187968849541, -322.6892615419374124 ) ) ;
#69622=CARTESIAN_POINT ( 'NONE',  ( -114.2397671894841977, -271.9008437961486493, -270.3528422294329516 ) ) ;
#69623=CARTESIAN_POINT ( 'NONE',  ( 3.677337364212458048, -274.7316543228658361, -331.9680378466097181 ) ) ;
#69624=CARTESIAN_POINT ( 'NONE',  ( -79.85767418267377593, -277.5519731276427251, -209.2570580049286662 ) ) ;
#69625=CARTESIAN_POINT ( 'NONE',  ( -110.5861565558097936, -273.8288976279920348, -264.8991047990763263 ) ) ;
#69626=CARTESIAN_POINT ( 'NONE',  ( -24.24262633470192441, -272.7908489176789999, -195.0277482228061672 ) ) ;
#69627=CARTESIAN_POINT ( 'NONE',  ( -110.3870821411951795, -297.8552413666325833, -279.6984704839471192 ) ) ;
#69629=CARTESIAN_POINT ( 'NONE',  ( -84.18605128844980356, -298.1918057863896365, -214.0970248975252730 ) ) ;
#69631=CARTESIAN_POINT ( 'NONE',  ( 20.21603067845342139, -286.2418557052944266, -318.9976724483742601 ) ) ;
#69632=CARTESIAN_POINT ( 'NONE',  ( -99.27935614528134067, -272.9187307297765983, -231.7252955946296993 ) ) ;
#69633=CARTESIAN_POINT ( 'NONE',  ( 31.42179433457710402, -287.1062884127480856, -235.7117048665498373 ) ) ;
#69634=CARTESIAN_POINT ( 'NONE',  ( -87.37391542011741308, -289.3942230992265650, -328.9334576981514147 ) ) ;
#69635=CARTESIAN_POINT ( 'NONE',  ( -110.6986872199104681, -298.3110318210101468, -287.6551597561391986 ) ) ;
#69636=CARTESIAN_POINT ( 'NONE',  ( 0.1387545234021022866, -292.5521961343963540, -335.1909533157337933 ) ) ;
#69637=CARTESIAN_POINT ( 'NONE',  ( 28.16198690622840672, -281.2763932557025441, -310.6294015380410656 ) ) ;
#69639=CARTESIAN_POINT ( 'NONE',  ( -110.2517982017299261, -276.3255934586799754, -287.9965871591145969 ) ) ;
#69641=CARTESIAN_POINT ( 'NONE',  ( -70.16373953786280993, -288.2894920572687738, -336.0244581608257022 ) ) ;
#69644=CARTESIAN_POINT ( 'NONE',  ( -86.00146978956946953, -287.7258796923047157, -327.5018115565001153 ) ) ;
#69645=CARTESIAN_POINT ( 'NONE',  ( -82.44901704040604784, -299.0249896612597809, -211.8859753007576785 ) ) ;
#69646=CARTESIAN_POINT ( 'NONE',  ( 19.35856810201305933, -283.6789760886103409, -321.6604785047875339 ) ) ;
#69647=CARTESIAN_POINT ( 'NONE',  ( -9.833932772768598340, -296.4149801694295547, -195.0151364894189783 ) ) ;
#69648=CARTESIAN_POINT ( 'NONE',  ( -45.63946840315497155, -283.1601082332524015, -342.9389832821836421 ) ) ;
#69649=CARTESIAN_POINT ( 'NONE',  ( -11.29854073748852983, -275.8233962234209002, -201.4798387571367755 ) ) ;
#69650=CARTESIAN_POINT ( 'NONE',  ( 20.41383522160819908, -282.8919155608105029, -222.5145006621147559 ) ) ;
#69651=CARTESIAN_POINT ( 'NONE',  ( -63.15120139018820566, -296.7664372253938723, -201.7707785825902533 ) ) ;
#69654=CARTESIAN_POINT ( 'NONE',  ( 38.85221289968654901, -293.2420205778114450, -258.8907986452902037 ) ) ;
#69655=CARTESIAN_POINT ( 'NONE',  ( -92.75890472143657917, -287.2330847048267515, -220.2773359872066123 ) ) ;
#69657=CARTESIAN_POINT ( 'NONE',  ( -88.47809603358389552, -276.9094976428775681, -206.1857440867352693 ) ) ;
#69658=CARTESIAN_POINT ( 'NONE',  ( -39.96769553396496377, -276.2814976625704162, -347.1677955074182478 ) ) ;
#69659=CARTESIAN_POINT ( 'NONE',  ( -74.05989551024291018, -287.9314525458897265, -337.1458795477659578 ) ) ;
#69660=CARTESIAN_POINT ( 'NONE',  ( -96.46654373640500069, -285.4610387780812175, -314.3493052856666736 ) ) ;
#69661=CARTESIAN_POINT ( 'NONE',  ( -10.87097574100657305, -278.4623477457084277, -339.4789504429181761 ) ) ;
#69662=CARTESIAN_POINT ( 'NONE',  ( -112.9075141173978807, -286.1246398783594032, -258.6796739838415533 ) ) ;
#69663=CARTESIAN_POINT ( 'NONE',  ( -13.41434335112037068, -281.5294584854959794, -339.8024156860477660 ) ) ;
#69664=CARTESIAN_POINT ( 'NONE',  ( -11.06568240610275566, -282.3946609979960840, -200.0596991083561136 ) ) ;
#69665=CARTESIAN_POINT ( 'NONE',  ( 38.21833966048116338, -275.5334665654639821, -255.5394989186387988 ) ) ;
#69666=CARTESIAN_POINT ( 'NONE',  ( -95.21219350160868089, -277.6981114264448820, -321.1548774538080124 ) ) ;
#69667=CARTESIAN_POINT ( 'NONE',  ( -9.937575162064501200, -296.6116357512788682, -339.5733144029186974 ) ) ;
#69668=CARTESIAN_POINT ( 'NONE',  ( 83.14890176555634582, -299.5541904835127980, -195.3611179825600175 ) ) ;
#69670=CARTESIAN_POINT ( 'NONE',  ( -76.46503071634499804, -293.7087191088846794, -335.3041377022019560 ) ) ;
#69671=CARTESIAN_POINT ( 'NONE',  ( 34.90344917153469595, -274.9151353466790511, -259.3852983307261866 ) ) ;
#69672=CARTESIAN_POINT ( 'NONE',  ( -54.53927079543026935, -298.9158327376727016, -195.6233358906989395 ) ) ;
#69674=CARTESIAN_POINT ( 'NONE',  ( -14.27112801539373166, -288.1154670088683929, -199.9815374597773427 ) ) ;
#69675=CARTESIAN_POINT ( 'NONE',  ( 36.74410336956815115, -294.8415629840635006, -252.0854107412757230 ) ) ;
#69676=CARTESIAN_POINT ( 'NONE',  ( -8.523104641325943476, -295.8884375453536677, -341.3926425442357413 ) ) ;
#69677=CARTESIAN_POINT ( 'NONE',  ( -99.62271437473184221, -291.9902192122026463, -311.8706216163864724 ) ) ;
#69678=CARTESIAN_POINT ( 'NONE',  ( -52.16623650159320391, -277.8619052757045438, -196.9578252153829112 ) ) ;
#69679=CARTESIAN_POINT ( 'NONE',  ( -82.17425835166110915, -281.3558445059095448, -210.8711644329430328 ) ) ;
#69680=CARTESIAN_POINT ( 'NONE',  ( -95.92148516596157037, -293.9968807049316979, -316.2928389022232523 ) ) ;
#69681=CARTESIAN_POINT ( 'NONE',  ( -47.07385096831357174, -285.0349398392034459, -345.4982640485495722 ) ) ;
#69682=CARTESIAN_POINT ( 'NONE',  ( -17.07327560764743524, -285.2402436463423214, -199.8565208904225869 ) ) ;
#69683=CARTESIAN_POINT ( 'NONE',  ( 140.7145785738311190, 179.0119726656982948, -240.7059938076026810 ) ) ;
#69685=CARTESIAN_POINT ( 'NONE',  ( -106.5509906701777254, -284.5299675815555815, -246.9184543612367975 ) ) ;
#69687=CARTESIAN_POINT ( 'NONE',  ( 30.80877462431995184, -283.0869971024856682, -305.5322041175897425 ) ) ;
#69688=CARTESIAN_POINT ( 'NONE',  ( -87.35087383678710182, -273.6650275178095626, -217.0831439453279472 ) ) ;
#69689=CARTESIAN_POINT ( 'NONE',  ( 21.79348265963942310, -285.6894941389752489, -221.6678034844456704 ) ) ;
#69690=CARTESIAN_POINT ( 'NONE',  ( -42.42647329689301472, -280.9307424363087193, -193.7649999679019004 ) ) ;
#69692=CARTESIAN_POINT ( 'NONE',  ( -96.29425163230303042, -280.7291436615811335, -221.8918057071531393 ) ) ;
#69693=CARTESIAN_POINT ( 'NONE',  ( 10.75278474919325333, -281.3482827075806085, -210.2909291872242932 ) ) ;
#69694=CARTESIAN_POINT ( 'NONE',  ( 27.33386217378598815, -279.4809262143061233, -301.5434626090942629 ) ) ;
#69695=CARTESIAN_POINT ( 'NONE',  ( -30.22131228085657639, -124.8493855615479333, -364.3862406674347199 ) ) ;
#69697=CARTESIAN_POINT ( 'NONE',  ( -86.53402864263458127, -275.3675513896361053, -213.8992736380239990 ) ) ;
#69698=CARTESIAN_POINT ( 'NONE',  ( 120.9473390240897288, 149.8309046525662893, -263.2900624566332226 ) ) ;
#69699=CARTESIAN_POINT ( 'NONE',  ( -65.41177754630301422, -277.7034775900432351, -201.1952480933589413 ) ) ;
#69700=CARTESIAN_POINT ( 'NONE',  ( 38.69757052014190890, -295.3113703493651769, -270.2882595025219530 ) ) ;
#69701=CARTESIAN_POINT ( 'NONE',  ( -45.10980184938776461, -294.5015661975689341, -343.0996922841786727 ) ) ;
#69702=CARTESIAN_POINT ( 'NONE',  ( -58.91541727020166519, -291.2879546567882016, -196.5092281506078677 ) ) ;
#69703=DIRECTION ( 'NONE',  ( -1.000000000000000000, 0.000000000000000000, -0.000000000000000000 ) ) ;
#69704=CARTESIAN_POINT ( 'NONE',  ( -109.2898969542203673, -295.4541939790075844, -244.6305279094046909 ) ) ;
#69705=CARTESIAN_POINT ( 'NONE',  ( 35.30564598893961659, -286.1215541422685646, -283.3535588046161138 ) ) ;
#69706=CARTESIAN_POINT ( 'NONE',  ( 20.28998939379037836, -294.7613150818826284, -223.5494216139058210 ) ) ;
#69707=CARTESIAN_POINT ( 'NONE',  ( -91.09077897360390352, -285.1513321543326356, -320.4837675685347449 ) ) ;
#69709=CARTESIAN_POINT ( 'NONE',  ( -101.4939421476263703, -292.0503621357454449, -228.1075531587300702 ) ) ;
#69710=CARTESIAN_POINT ( 'NONE',  ( -26.72764481270809966, -283.4059881267299943, -342.6989074079527882 ) ) ;
#69711=CARTESIAN_POINT ( 'NONE',  ( -97.96965203886895779, -294.7188887277228559, -317.1826959917278259 ) ) ;
#69712=CARTESIAN_POINT ( 'NONE',  ( -78.04218483948140772, -290.3868880944109492, -335.5970198268556715 ) ) ;
#69713=CARTESIAN_POINT ( 'NONE',  ( -70.87655904692489628, -292.1138578350687567, -201.1156116959616895 ) ) ;
#69714=CARTESIAN_POINT ( 'NONE',  ( 18.66039553679151197, -287.0539705062516305, -223.5146725238399767 ) ) ;
#69717=CARTESIAN_POINT ( 'NONE',  ( -71.49567081594838669, -297.3588689817902377, -337.9910800560779194 ) ) ;
#69718=CARTESIAN_POINT ( 'NONE',  ( -96.95151132392916793, -295.8838805124827331, -222.4031292392906494 ) ) ;
#69719=CARTESIAN_POINT ( 'NONE',  ( -24.82442774050839063, -279.2745142269370717, -198.2034687728357483 ) ) ;
#69721=CARTESIAN_POINT ( 'NONE',  ( -15.78858267145959893, -273.8312352855726886, -196.4479173958833371 ) ) ;
#69722=CARTESIAN_POINT ( 'NONE',  ( -67.08155842100754285, -296.1349592835214253, -202.9214354106515259 ) ) ;
#69723=CARTESIAN_POINT ( 'NONE',  ( -6.981167555458131169, -278.5098615126699997, -338.1040404523436678 ) ) ;
#69724=CARTESIAN_POINT ( 'NONE',  ( 20.83809819108577699, -273.0515670545426019, -224.2324558410964528 ) ) ;
#69725=CARTESIAN_POINT ( 'NONE',  ( 8.488007922102811520, -295.6137809593959673, -327.7567921259814057 ) ) ;
#69726=CARTESIAN_POINT ( 'NONE',  ( -70.62010500271038893, -298.6822962338720231, -205.0265995652705158 ) ) ;
#69728=CARTESIAN_POINT ( 'NONE',  ( -65.26799606271249843, -299.2934514397364865, -199.4064600910867568 ) ) ;
#69729=CARTESIAN_POINT ( 'NONE',  ( -62.21381125162950099, -295.7292613181587058, -199.4287099186476269 ) ) ;
#69730=CARTESIAN_POINT ( 'NONE',  ( -75.03927471209844668, -292.1873619957120241, -207.6698719003199471 ) ) ;
#69731=CARTESIAN_POINT ( 'NONE',  ( -99.34794368747793669, -288.5831111782462699, -309.9919226229670244 ) ) ;
#69733=CARTESIAN_POINT ( 'NONE',  ( -29.85111695228361484, -274.6369201365360482, -193.7881588725065285 ) ) ;
#69735=CARTESIAN_POINT ( 'NONE',  ( -108.1964937790721848, -297.1189531061372691, -252.6552924405738167 ) ) ;
#69737=CARTESIAN_POINT ( 'NONE',  ( -25.67563479675024496, -282.1799768831593269, -195.9144275247023472 ) ) ;
#69738=CARTESIAN_POINT ( 'NONE',  ( 28.86823909258136922, -279.7352672738903721, -232.0265093353434622 ) ) ;
#69739=CARTESIAN_POINT ( 'NONE',  ( -20.15696530941892561, -276.1856649388651590, -345.3690662258242128 ) ) ;
#69740=CARTESIAN_POINT ( 'NONE',  ( 30.48040363235761774, -281.1159244179107191, -297.7976623725783725 ) ) ;
#69741=CARTESIAN_POINT ( 'NONE',  ( 30.72124011757808049, -279.9718200221510642, -302.3813783619380615 ) ) ;
#69742=CARTESIAN_POINT ( 'NONE',  ( -79.17523822138906553, -272.0504809732748868, -209.7572605347168349 ) ) ;
#69743=CARTESIAN_POINT ( 'NONE',  ( -107.8859270491339544, -280.2204198855991990, -295.9764994671540421 ) ) ;
#69746=CARTESIAN_POINT ( 'NONE',  ( -111.0392422152190335, -271.1993468556269136, -250.7915491121219134 ) ) ;
#69748=CARTESIAN_POINT ( 'NONE',  ( 34.32260354411413061, -277.8442825706679855, -293.0383313444550026 ) ) ;
#69749=CARTESIAN_POINT ( 'NONE',  ( -63.99428340552925931, -271.7044068883166688, -200.2427601859610888 ) ) ;
#69751=CARTESIAN_POINT ( 'NONE',  ( -96.03801923425133680, -285.8217034560387901, -317.9635441034330938 ) ) ;
#69754=CARTESIAN_POINT ( 'NONE',  ( 36.49117538660233606, -285.7248481210004911, -283.8235244442412863 ) ) ;
#69756=CARTESIAN_POINT ( 'NONE',  ( 33.82734164008455480, -292.5826543758534513, -288.3082068760462562 ) ) ;
#69757=CARTESIAN_POINT ( 'NONE',  ( 29.32684438253895465, -286.1266864253406084, -303.0133866673531884 ) ) ;
#69758=CARTESIAN_POINT ( 'NONE',  ( 0.9968329295543288948, -56.25428601379442028, -352.6033083298257225 ) ) ;
#69759=CARTESIAN_POINT ( 'NONE',  ( -89.92166824827005200, -293.7939382230401861, -323.9163461860904931 ) ) ;
#69760=CARTESIAN_POINT ( 'NONE',  ( -103.4301990598390404, -283.5336362849516263, -232.1113863837517499 ) ) ;
#69761=CARTESIAN_POINT ( 'NONE',  ( -37.02512560537597608, -281.6563111726727584, -196.5617941490830844 ) ) ;
#69762=CARTESIAN_POINT ( 'NONE',  ( 38.39067834454567674, -288.6113591915424195, -258.7580135312788343 ) ) ;
#69763=CARTESIAN_POINT ( 'NONE',  ( 25.08486774103853634, -280.3722526985122840, -313.7071694180844474 ) ) ;
#69764=CARTESIAN_POINT ( 'NONE',  ( -98.84176588497294347, -290.0081536835057250, -309.6897578255295116 ) ) ;
#69765=CARTESIAN_POINT ( 'NONE',  ( -41.09927852052798158, -281.4292099863754970, -196.8678834459775260 ) ) ;
#69766=CARTESIAN_POINT ( 'NONE',  ( -49.17808029720806928, -280.7002758255341064, -198.1634599108560906 ) ) ;
#69767=CARTESIAN_POINT ( 'NONE',  ( 35.20785125506043300, -289.7934350737350542, -290.7792948705354661 ) ) ;
#69770=CARTESIAN_POINT ( 'NONE',  ( -114.3417001280813849, -272.5880137785256352, -267.4936526912260319 ) ) ;
#69771=CARTESIAN_POINT ( 'NONE',  ( -73.12569881047713238, -291.5089085225822600, -335.8695315084829645 ) ) ;
#69773=CARTESIAN_POINT ( 'NONE',  ( -2.602324593224680793, -297.1233781216987495, -342.4248175857292154 ) ) ;
#69774=VERTEX_POINT ( 'NONE', #15127 ) ;
#69775=CARTESIAN_POINT ( 'NONE',  ( 15.64437633638226721, -274.3048549049173062, -323.7489116557920283 ) ) ;
#69776=FACE_OUTER_BOUND ( 'NONE', #12896, .T. ) ;
#69777=CARTESIAN_POINT ( 'NONE',  ( -58.64738260790357316, -293.7229202153291112, -343.5769557234759759 ) ) ;
#69778=CARTESIAN_POINT ( 'NONE',  ( -102.5844659797832179, -296.5071070721870683, -237.3643002194833116 ) ) ;
#69779=CARTESIAN_POINT ( 'NONE',  ( 14.58552900387998719, -289.8249363724557952, -322.6513716293845846 ) ) ;
#69780=CARTESIAN_POINT ( 'NONE',  ( 10.58165542477711973, -284.1400506273893143, -326.8317791075056675 ) ) ;
#69781=CARTESIAN_POINT ( 'NONE',  ( -91.17045695381112580, -291.2239468179803907, -324.6671753163211065 ) ) ;
#69782=CARTESIAN_POINT ( 'NONE',  ( -104.7137327352939735, -291.3955604553779040, -306.6144970512342525 ) ) ;
#69783=CARTESIAN_POINT ( 'NONE',  ( -72.12786754061581007, -287.5921755839538605, -203.9162294783904770 ) ) ;
#69784=CARTESIAN_POINT ( 'NONE',  ( -8.863084547796210799, -280.5812610166687477, -198.8211399343347807 ) ) ;
#69785=CARTESIAN_POINT ( 'NONE',  ( -101.8982269055259593, -294.1095378964258771, -309.6264849986258128 ) ) ;
#69786=CARTESIAN_POINT ( 'NONE',  ( -41.57126057071925374, -282.9372209981283390, -347.2971932153177477 ) ) ;
#69787=CARTESIAN_POINT ( 'NONE',  ( 14.33988895547520492, -276.6485737450211673, -217.0706044863480315 ) ) ;
#69788=CARTESIAN_POINT ( 'NONE',  ( 34.45848030099739390, -284.0519495502702512, -270.3284710469131937 ) ) ;
#69789=CARTESIAN_POINT ( 'NONE',  ( 37.73100448102987770, -273.9451015590176439, -282.4407652439108460 ) ) ;
#69791=CARTESIAN_POINT ( 'NONE',  ( -7.968956325360199600, -279.9552851650930734, -203.4502708190228759 ) ) ;
#69792=CARTESIAN_POINT ( 'NONE',  ( -113.3701832252194919, -279.6342411833419419, -280.1440915724574552 ) ) ;
#69793=CARTESIAN_POINT ( 'NONE',  ( -57.68201391988490911, -284.8546305326102015, -196.2850499678423262 ) ) ;
#69794=CARTESIAN_POINT ( 'NONE',  ( 20.96755605993838856, -294.6782807176982146, -224.7554711247354362 ) ) ;
#69795=CARTESIAN_POINT ( 'NONE',  ( 36.46896285214925371, -277.3916859713029908, -289.2932717934054949 ) ) ;
#69796=CARTESIAN_POINT ( 'NONE',  ( -46.83650365200139021, -275.2491525289918286, -194.4457244313477418 ) ) ;
#69798=CARTESIAN_POINT ( 'NONE',  ( 9.662428170168167796, -276.2172169285096288, -326.2146042426433041 ) ) ;
#69799=CARTESIAN_POINT ( 'NONE',  ( -81.20940412451946600, -297.6500928145194393, -330.9882816124076612 ) ) ;
#69800=CARTESIAN_POINT ( 'NONE',  ( -84.79114728922037614, -283.3965685785242954, -212.4269057746222131 ) ) ;
#69801=CARTESIAN_POINT ( 'NONE',  ( 39.69046493787777052, -293.2182848010341445, -270.3142089617036845 ) ) ;
#69802=CARTESIAN_POINT ( 'NONE',  ( 36.47184717657550124, -273.4278304277079314, -259.1660536005069275 ) ) ;
#69803=CARTESIAN_POINT ( 'NONE',  ( 37.99155650847939825, -289.0063480829616083, -258.8139895386072453 ) ) ;
#69804=CARTESIAN_POINT ( 'NONE',  ( -37.53702834384171894, -290.9700129800380637, -197.0397683845907579 ) ) ;
#69806=CARTESIAN_POINT ( 'NONE',  ( -61.48506261730522482, -290.3194146842748751, -197.8091588838541952 ) ) ;
#69807=CARTESIAN_POINT ( 'NONE',  ( -110.1440873523407049, -290.1362289151088021, -276.6274992141105713 ) ) ;
#69808=ORIENTED_EDGE ( 'NONE', *, *, #33448, .F. ) ;
#69809=CARTESIAN_POINT ( 'NONE',  ( 21.84282116196428092, -287.9738715971319607, -221.5893541155373043 ) ) ;
#69810=CARTESIAN_POINT ( 'NONE',  ( -107.8395674423771453, -278.6341407871074694, -289.3910468046250912 ) ) ;
#69811=CARTESIAN_POINT ( 'NONE',  ( -90.50773146999405583, -294.7039969918437805, -325.7050836276022210 ) ) ;
#69812=CARTESIAN_POINT ( 'NONE',  ( -2.276798263768706754, -287.1552592888003232, -201.9083446490197389 ) ) ;
#69813=CARTESIAN_POINT ( 'NONE',  ( 26.33748730263272719, -287.3147461526577331, -227.0859209131998568 ) ) ;
#69814=CARTESIAN_POINT ( 'NONE',  ( -1.237861536918885674, -282.8922144017213895, -333.8323738846017932 ) ) ;
#69815=CARTESIAN_POINT ( 'NONE',  ( -84.14657331821624098, -219.4986398962294913, -352.5341896374943644 ) ) ;
#69817=CARTESIAN_POINT ( 'NONE',  ( 23.98614183410543532, -22.50930313572179031, -343.8471797293080954 ) ) ;
#69818=CARTESIAN_POINT ( 'NONE',  ( -94.70623550478640595, -238.3196911832316687, -338.6262115470744334 ) ) ;
#69819=CIRCLE ( 'NONE', #25934, 5.654241149514405151 ) ;
#69820=CARTESIAN_POINT ( 'NONE',  ( 35.51388148748905138, -274.8372838068893316, -277.0443772284637589 ) ) ;
#69821=CARTESIAN_POINT ( 'NONE',  ( 33.53755888985122624, -274.7186001613494568, -289.0789361095579579 ) ) ;
#69822=CARTESIAN_POINT ( 'NONE',  ( -57.36765198758669015, -297.3082056036287781, -196.0193574158977867 ) ) ;
#69823=CARTESIAN_POINT ( 'NONE',  ( 7.158040960647978679, -59.91464807905658319, -351.6596033274320234 ) ) ;
#69824=CARTESIAN_POINT ( 'NONE',  ( 21.48249569608899989, -273.5748194817562080, -221.4426934365206705 ) ) ;
#69825=CARTESIAN_POINT ( 'NONE',  ( -27.17283030142132816, -275.9431733507386184, -196.9980682311274904 ) ) ;
#69827=CARTESIAN_POINT ( 'NONE',  ( -112.0739693511602724, -297.2725598971451859, -287.9652485549684116 ) ) ;
#69828=CARTESIAN_POINT ( 'NONE',  ( 1.349481396886883289, -289.0122455190566484, -332.3367657308255048 ) ) ;
#69829=CARTESIAN_POINT ( 'NONE',  ( -109.2827416163746364, -297.0111148477424194, -297.5046112250822716 ) ) ;
#69830=CARTESIAN_POINT ( 'NONE',  ( -113.0796440280699642, -297.2139501283534173, -256.8226262959033761 ) ) ;
#69831=CARTESIAN_POINT ( 'NONE',  ( 24.84675797149762744, -293.1906821969593011, -232.0343378902414031 ) ) ;
#69832=EDGE_LOOP ( 'NONE', ( #53142, #85059, #21411, #84841 ) ) ;
#69833=CARTESIAN_POINT ( 'NONE',  ( 34.69726164150895187, -277.7642890607971253, -293.1580955276006648 ) ) ;
#69836=CARTESIAN_POINT ( 'NONE',  ( 17.18392958689692662, -280.3120479773417628, -216.0048937307164181 ) ) ;
#69837=CARTESIAN_POINT ( 'NONE',  ( -68.12544915272330570, -278.4078514846190728, -336.8261632510392474 ) ) ;
#69838=CARTESIAN_POINT ( 'NONE',  ( -35.71049021314031080, -278.7921205503171223, -346.3432279159363247 ) ) ;
#69839=CARTESIAN_POINT ( 'NONE',  ( -93.99130473467940305, -275.8851922394803751, -320.0524562882885675 ) ) ;
#69840=CARTESIAN_POINT ( 'NONE',  ( -70.52121750823587831, -298.2541073234322653, -205.2087775785396389 ) ) ;
#69841=CARTESIAN_POINT ( 'NONE',  ( -110.9739623088040190, -295.1125720020813787, -271.4538989148142605 ) ) ;
#69843=CARTESIAN_POINT ( 'NONE',  ( -4.975584933748663730, -280.9593298086963955, -200.5616803720582766 ) ) ;
#69844=EDGE_CURVE ( 'NONE', #65957, #62648, #14498, .T. ) ;
#69845=CARTESIAN_POINT ( 'NONE',  ( -107.8197076371699978, -278.4675665788223569, -289.3834853975744750 ) ) ;
#69846=CARTESIAN_POINT ( 'NONE',  ( 32.40837223325540606, -286.6411257774357182, -301.7971749401472152 ) ) ;
#69847=CARTESIAN_POINT ( 'NONE',  ( -36.58988087788193155, -300.0616984865663426, -195.1941870151826492 ) ) ;
#69849=CARTESIAN_POINT ( 'NONE',  ( -108.5098687401455777, -289.5260411048391802, -287.3226481003029562 ) ) ;
#69850=CARTESIAN_POINT ( 'NONE',  ( -62.63445947834218686, -277.9584268299190626, -200.7494947566690939 ) ) ;
#69851=CARTESIAN_POINT ( 'NONE',  ( -16.73950341344101389, -278.8982833906938481, -199.7146431497733090 ) ) ;
#69852=CARTESIAN_POINT ( 'NONE',  ( -62.03502070899428844, -281.4554058552522520, -340.6404367515655736 ) ) ;
#69853=CARTESIAN_POINT ( 'NONE',  ( 35.13370030931157117, -289.3020423786359743, -250.8717609994892257 ) ) ;
#69854=CARTESIAN_POINT ( 'NONE',  ( -110.2969430991380051, -279.6458451373547405, -278.8509030828682853 ) ) ;
#69856=CARTESIAN_POINT ( 'NONE',  ( 16.04752219468317520, -294.8088544809635323, -217.6136231182229039 ) ) ;
#69857=CARTESIAN_POINT ( 'NONE',  ( -95.38978219616744525, -276.1224197385801631, -319.4158308149458207 ) ) ;
#69858=CARTESIAN_POINT ( 'NONE',  ( 7.649648561228860721, -277.0710919898075417, -328.0422134411126081 ) ) ;
#69859=CARTESIAN_POINT ( 'NONE',  ( -34.52162790334747200, -285.0169364510393279, -345.4748691988879727 ) ) ;
#69860=DIRECTION ( 'NONE',  ( 0.000000000000000000, 0.000000000000000000, 1.000000000000000000 ) ) ;
#69861=CARTESIAN_POINT ( 'NONE',  ( -110.9207199349052360, -292.6913679100433114, -253.1726902823849912 ) ) ;
#69862=CARTESIAN_POINT ( 'NONE',  ( -50.59282230630184074, -293.2210865090200969, -344.2334130830394656 ) ) ;
#69863=CARTESIAN_POINT ( 'NONE',  ( 1.449007683615202380, -285.7538595798659458, -204.0175376582806734 ) ) ;
#69865=CARTESIAN_POINT ( 'NONE',  ( -56.97736901219635541, -272.4784976865049089, -199.4865550070201436 ) ) ;
#69866=CARTESIAN_POINT ( 'NONE',  ( -0.6254859487067386814, -290.6850126336611311, -205.8267465246558743 ) ) ;
#69869=CARTESIAN_POINT ( 'NONE',  ( -98.63600406859396230, -289.6420105566908774, -224.8890871053053786 ) ) ;
#69870=CARTESIAN_POINT ( 'NONE',  ( -71.56712800353275838, -287.1922081489394714, -204.9771711487841799 ) ) ;
#69871=CARTESIAN_POINT ( 'NONE',  ( 38.59052326206262507, -285.8430928982788828, -274.3918300862579827 ) ) ;
#69872=CARTESIAN_POINT ( 'NONE',  ( -105.7550710406451913, -285.6160272760651537, -297.6103601237347789 ) ) ;
#69874=CARTESIAN_POINT ( 'NONE',  ( -101.1371230449171890, -285.8451928693472155, -234.4418291461244337 ) ) ;
#69875=CARTESIAN_POINT ( 'NONE',  ( 18.18621742184801349, -294.8238034799593947, -219.4194142803737861 ) ) ;
#69876=CARTESIAN_POINT ( 'NONE',  ( 17.83465341282682814, -274.3495558591986310, -321.9836344663979730 ) ) ;
#69877=CARTESIAN_POINT ( 'NONE',  ( 31.83814585659040830, -276.3204113725470279, -304.2448489721358555 ) ) ;
#69879=CARTESIAN_POINT ( 'NONE',  ( -58.51136796910393656, -289.8603776747629581, -197.8272682355132019 ) ) ;
#69880=CARTESIAN_POINT ( 'NONE',  ( -69.96237619135595764, -279.6343191865573772, -200.5979545221962042 ) ) ;
#69881=CARTESIAN_POINT ( 'NONE',  ( -76.49991774877359774, -297.5582207467612079, -333.9704102226644977 ) ) ;
#69883=CARTESIAN_POINT ( 'NONE',  ( 129.8975571001389540, -299.5541904835127980, -195.3611179825600175 ) ) ;
#69884=CARTESIAN_POINT ( 'NONE',  ( -6.796362452137638677, -285.1465249386672554, -203.5025076557707564 ) ) ;
#69885=CARTESIAN_POINT ( 'NONE',  ( 17.70989211536642927, -278.8397325102552031, -219.4266223947996650 ) ) ;
#69887=CARTESIAN_POINT ( 'NONE',  ( 36.96423561809814373, -273.8123132421795276, -252.9451924945206827 ) ) ;
#69888=CARTESIAN_POINT ( 'NONE',  ( -100.6752867818674986, -277.3996614920042703, -306.9696441423736246 ) ) ;
#69890=CARTESIAN_POINT ( 'NONE',  ( -15.36780548047465089, -296.2827437851610171, -340.7557947926619022 ) ) ;
#69891=CARTESIAN_POINT ( 'NONE',  ( 37.83979153515001315, -280.6626022124785891, -285.5016537083496928 ) ) ;
#69892=CARTESIAN_POINT ( 'NONE',  ( -5.428173927389670972, -295.5629120734810158, -336.2910976143267021 ) ) ;
#69893=CARTESIAN_POINT ( 'NONE',  ( -68.01300627710857327, -296.7616748436985858, -340.4508408597426410 ) ) ;
#69894=CARTESIAN_POINT ( 'NONE',  ( -60.51388748766771641, -297.5765301800841485, -201.0830169799158682 ) ) ;
#69895=CARTESIAN_POINT ( 'NONE',  ( -91.27168227241885745, -293.2853276991085067, -218.2405109806711039 ) ) ;
#69896=CARTESIAN_POINT ( 'NONE',  ( -68.50270329652708767, -285.8205997747404581, -199.9337321232605404 ) ) ;
#69897=CARTESIAN_POINT ( 'NONE',  ( 37.27975156300217918, -273.5241291862529920, -257.1740976037683595 ) ) ;
#69898=CARTESIAN_POINT ( 'NONE',  ( -41.76267913961567757, -288.9396937276749782, -347.2473194799576390 ) ) ;
#69899=CARTESIAN_POINT ( 'NONE',  ( -111.9970392151001874, -280.5640829750805665, -267.8781502151322798 ) ) ;
#69900=CARTESIAN_POINT ( 'NONE',  ( 22.18982810042686182, -286.0156232565913683, -227.6211106795291244 ) ) ;
#69901=CARTESIAN_POINT ( 'NONE',  ( -110.0492601287574672, -288.7889813451972145, -251.9080641120842756 ) ) ;
#69902=CARTESIAN_POINT ( 'NONE',  ( -47.20788896421541381, -156.8319029772612225, -362.3615984655540387 ) ) ;
#69903=CARTESIAN_POINT ( 'NONE',  ( 35.61450233827622469, -286.9969017672466975, -265.5889255935906021 ) ) ;
#69905=CARTESIAN_POINT ( 'NONE',  ( -52.85829936820156405, -284.1874453095255717, -345.5955943772180490 ) ) ;
#69906=CARTESIAN_POINT ( 'NONE',  ( -58.86120577092684414, -290.8391221403008444, -196.6744089417883856 ) ) ;
#69907=CARTESIAN_POINT ( 'NONE',  ( 38.38533278721116204, -283.0393257420132045, -261.4233548760137751 ) ) ;
#69908=CARTESIAN_POINT ( 'NONE',  ( 39.21686377178659200, -282.8617261796161415, -269.9163106681361910 ) ) ;
#69909=CARTESIAN_POINT ( 'NONE',  ( 35.56581522207419965, -281.4339299176273244, -274.0345645865812685 ) ) ;
#69910=CARTESIAN_POINT ( 'NONE',  ( 36.81545282730818514, -277.4072407561739624, -259.0625264375866550 ) ) ;
#69911=CARTESIAN_POINT ( 'NONE',  ( -30.59095141396967676, -294.9690163808668331, -347.0646211085511368 ) ) ;
#69912=CARTESIAN_POINT ( 'NONE',  ( -110.2751125260875114, -288.3665244729839401, -286.3128998105893857 ) ) ;
#69914=CARTESIAN_POINT ( 'NONE',  ( -44.58600641714774326, -296.8787991150953189, -197.3602239962473277 ) ) ;
#69915=ORIENTED_EDGE ( 'NONE', *, *, #69844, .T. ) ;
#69917=CARTESIAN_POINT ( 'NONE',  ( -108.7430303059190919, -286.7475585476391871, -249.1306703359411472 ) ) ;
#69918=CARTESIAN_POINT ( 'NONE',  ( 36.40312563877686358, -294.3663138658903904, -249.2611441561102765 ) ) ;
#69919=CARTESIAN_POINT ( 'NONE',  ( -13.48827728622425681, -283.3856482824953105, -339.5155007035441486 ) ) ;
#69920=CARTESIAN_POINT ( 'NONE',  ( 29.74774395412104511, -274.1245982420526275, -232.9445877546250472 ) ) ;
#69921=CARTESIAN_POINT ( 'NONE',  ( -103.1329390377102868, -291.7249831284295851, -230.4485663156505950 ) ) ;
#69922=CARTESIAN_POINT ( 'NONE',  ( -29.56577140520561997, -284.2892252297237405, -194.9964020195030230 ) ) ;
#69923=CARTESIAN_POINT ( 'NONE',  ( 1.685719059630385042, -292.8919950087804409, -203.9480751310505013 ) ) ;
#69924=CARTESIAN_POINT ( 'NONE',  ( 19.53262534828831676, -288.5327328133406581, -316.1584824098508761 ) ) ;
#69926=DIRECTION ( 'NONE',  ( 0.000000000000000000, 0.000000000000000000, -1.000000000000000000 ) ) ;
#69927=CARTESIAN_POINT ( 'NONE',  ( 196.4392320932925600, 281.7853120024273608, -110.2283348974790869 ) ) ;
#69928=CARTESIAN_POINT ( 'NONE',  ( -78.76694709226494240, -285.1196251605589396, -334.4443191011737895 ) ) ;
#69929=CARTESIAN_POINT ( 'NONE',  ( 10.59707575819633618, -285.9094976428776818, -330.5268031993606428 ) ) ;
#69931=CARTESIAN_POINT ( 'NONE',  ( 35.34111816847146059, -280.3419028635861991, -260.4210565170488962 ) ) ;
#69932=CARTESIAN_POINT ( 'NONE',  ( 14.86572119087143129, -276.0071912240183565, -327.0033499816094036 ) ) ;
#69933=CARTESIAN_POINT ( 'NONE',  ( -110.4020798630876641, -280.7613765721303594, -254.1094854745516329 ) ) ;
#69934=CARTESIAN_POINT ( 'NONE',  ( -109.3818371394523439, -271.0219980206236414, -295.8620562373184271 ) ) ;
#69935=CARTESIAN_POINT ( 'NONE',  ( 37.28609729605216927, -280.3344632765735014, -286.8317849141425881 ) ) ;
#69936=CARTESIAN_POINT ( 'NONE',  ( -52.39657739801258884, -283.8784975105800186, -197.2502605808462590 ) ) ;
#69937=CARTESIAN_POINT ( 'NONE',  ( -65.19176344665378053, -299.4534384573961461, -199.6058755778817613 ) ) ;
#69938=CARTESIAN_POINT ( 'NONE',  ( 19.74577498377869844, -294.6882289870004570, -315.9772112643364608 ) ) ;
#69940=CARTESIAN_POINT ( 'NONE',  ( -62.95702436984655748, -290.3963097146722134, -201.4764415882426647 ) ) ;
#69941=CARTESIAN_POINT ( 'NONE',  ( -42.79065688494367947, -277.7706278094759682, -347.0658874359046990 ) ) ;
#69942=CARTESIAN_POINT ( 'NONE',  ( -38.08236020527431975, -274.0426155692717884, -197.3648754583721256 ) ) ;
#69943=CARTESIAN_POINT ( 'NONE',  ( -112.7617452633776907, -271.6506261557143489, -256.1742905084807376 ) ) ;
#69945=CARTESIAN_POINT ( 'NONE',  ( 5.292311968802505540, -272.6283614942753388, -208.5950628434527232 ) ) ;
#69950=CARTESIAN_POINT ( 'NONE',  ( 20.43304003651921619, -283.2651762691130557, -315.4865595157622238 ) ) ;
#69951=CARTESIAN_POINT ( 'NONE',  ( 29.81559632849957353, -282.8457929027379123, -234.6980312739503631 ) ) ;
#69952=CARTESIAN_POINT ( 'NONE',  ( -87.00416110652288637, -283.1139222855458684, -324.0730167631756444 ) ) ;
#69953=CARTESIAN_POINT ( 'NONE',  ( -0.1254269126662794498, -272.9559501441321459, -206.6173338480240318 ) ) ;
#69954=CARTESIAN_POINT ( 'NONE',  ( -27.41629240917883692, -282.0398738299962247, -196.7403753057948563 ) ) ;
#69955=CARTESIAN_POINT ( 'NONE',  ( 33.17424939053778132, -274.3133206007054241, -291.8106313566112817 ) ) ;
#69958=CARTESIAN_POINT ( 'NONE',  ( 34.13206991952225877, -276.4170298106874384, -254.0039281962677080 ) ) ;
#69961=CARTESIAN_POINT ( 'NONE',  ( -17.38995559178933803, -277.6038541676886098, -344.5641280965680266 ) ) ;
#69965=CARTESIAN_POINT ( 'NONE',  ( -64.13293707563521195, -287.5667750853426128, -199.4773295001671158 ) ) ;
#69966=CARTESIAN_POINT ( 'NONE',  ( -95.73938617503270621, -295.1313631101084525, -314.4534279047908285 ) ) ;
#69968=CARTESIAN_POINT ( 'NONE',  ( -20.52678491702211971, -288.1904135201629060, -345.4528450825957293 ) ) ;
#69969=CARTESIAN_POINT ( 'NONE',  ( -95.74301710409903876, -283.4241212034692126, -224.8734130622021041 ) ) ;
#69970=CARTESIAN_POINT ( 'NONE',  ( -109.2367046352238020, -283.3330946910367629, -254.6025676901048769 ) ) ;
#69971=CARTESIAN_POINT ( 'NONE',  ( -93.19092824606018155, -288.1083717983200927, -319.0056040404932673 ) ) ;
#69972=CARTESIAN_POINT ( 'NONE',  ( -80.84923534651552757, -284.8623111566564603, -329.5363113563394677 ) ) ;
#69973=CARTESIAN_POINT ( 'NONE',  ( 2.419046556365148426, -274.5195751371769006, -334.0153498427671366 ) ) ;
#69974=CARTESIAN_POINT ( 'NONE',  ( 33.12745311249031488, -285.5781770154042647, -241.2311322837780665 ) ) ;
#69975=CARTESIAN_POINT ( 'NONE',  ( -83.99282008578568082, -299.4112751593642088, -211.6357090669144725 ) ) ;
#69976=CARTESIAN_POINT ( 'NONE',  ( 28.73854083186291319, -286.0280141197459329, -306.2949013406263248 ) ) ;
#69977=CARTESIAN_POINT ( 'NONE',  ( -51.88577660282197002, -280.8028444406000403, -198.5326333571745465 ) ) ;
#69978=CARTESIAN_POINT ( 'NONE',  ( -26.38599813561156893, -290.9131880073628622, -344.7250945994023823 ) ) ;
#69981=CARTESIAN_POINT ( 'NONE',  ( -63.73976035961275954, -297.3138090366653046, -341.1598228694620616 ) ) ;
#69983=CARTESIAN_POINT ( 'NONE',  ( -27.26511985092312074, -278.1799192299293964, -195.9885173964854346 ) ) ;
#69984=CARTESIAN_POINT ( 'NONE',  ( 29.34059094481437668, -292.2522505028048272, -232.1821856066808039 ) ) ;
#69985=CARTESIAN_POINT ( 'NONE',  ( -110.8451493102328129, -295.0454339692290091, -263.2020036758684682 ) ) ;
#69986=CARTESIAN_POINT ( 'NONE',  ( 9.604337228643641922, -279.3982695602122135, -213.7499774159815900 ) ) ;
#69987=CARTESIAN_POINT ( 'NONE',  ( 29.15845152836323706, -273.1867841343486134, -236.9090025847019945 ) ) ;
#69988=CARTESIAN_POINT ( 'NONE',  ( 16.53196190812811395, -295.5809594945984600, -320.3498368810196553 ) ) ;
#69989=CARTESIAN_POINT ( 'NONE',  ( -69.91165696735023971, -294.1233781216987495, -202.8022627189028810 ) ) ;
#69990=CARTESIAN_POINT ( 'NONE',  ( -106.5457882174293616, -294.6168630523359866, -302.5092430074454342 ) ) ;
#69991=CARTESIAN_POINT ( 'NONE',  ( -25.16149338894066645, -290.4452738144798332, -195.3570075918393059 ) ) ;
#69992=CARTESIAN_POINT ( 'NONE',  ( -104.5787582552584638, -291.5765062153187159, -300.3959700923375067 ) ) ;
#69994=CARTESIAN_POINT ( 'NONE',  ( -105.8654724817034491, -291.6979189197457458, -244.5834585213102343 ) ) ;
#69996=CARTESIAN_POINT ( 'NONE',  ( -90.52138181916453163, -292.5244193230292922, -215.1519230775317055 ) ) ;
#69997=CARTESIAN_POINT ( 'NONE',  ( 36.52807747296611041, -279.7625270273228466, -285.2494611819862484 ) ) ;
#69998=CARTESIAN_POINT ( 'NONE',  ( 12.90315701401277337, -292.7776524292532372, -217.4040190177323666 ) ) ;
#69999=CARTESIAN_POINT ( 'NONE',  ( 15.16133415868702983, -280.7686147112395929, -213.9638891745606486 ) ) ;
#70000=CARTESIAN_POINT ( 'NONE',  ( -88.31071586364588200, -283.4097281426055588, -328.1202810978776370 ) ) ;
#70001=CARTESIAN_POINT ( 'NONE',  ( -98.87046001399515660, -287.9728612838627555, -312.9775389237487389 ) ) ;
#70002=CARTESIAN_POINT ( 'NONE',  ( -51.27253721878857107, -281.3715667942249183, -343.3299413249704344 ) ) ;
#70003=CARTESIAN_POINT ( 'NONE',  ( -79.51135550676674768, -277.9739975718666756, -206.7019273469587688 ) ) ;
#70004=CARTESIAN_POINT ( 'NONE',  ( -4.892191116106971549, -285.3898590538238977, -200.8735516413862285 ) ) ;
#70006=CARTESIAN_POINT ( 'NONE',  ( 0.2997534686382283264, -294.1627103920170043, -206.8822916992624528 ) ) ;
#70007=CARTESIAN_POINT ( 'NONE',  ( 12.33541055560685784, -277.8012915519076387, -328.4196312728062708 ) ) ;
#70008=CARTESIAN_POINT ( 'NONE',  ( -103.1519066630730919, -277.7895283523055809, -302.1183613250405529 ) ) ;
#70009=CARTESIAN_POINT ( 'NONE',  ( -61.69059341658992679, -291.9111105554095502, -197.2561316515332237 ) ) ;
#70011=CARTESIAN_POINT ( 'NONE',  ( 20.49177049563761699, -280.2992811304096108, -318.9883107528715414 ) ) ;
#70012=CARTESIAN_POINT ( 'NONE',  ( 32.02776521367444218, -292.2980601191121082, -246.7237024695453442 ) ) ;
#70013=CIRCLE ( 'NONE', #82090, 2.738891987356051327 ) ;
#70014=CARTESIAN_POINT ( 'NONE',  ( -96.63668418683886330, -295.1817193960060308, -224.4154023411693402 ) ) ;
#70018=CARTESIAN_POINT ( 'NONE',  ( 34.38359394569770444, -293.2431364434484635, -284.2704900693136096 ) ) ;
#70020=CARTESIAN_POINT ( 'NONE',  ( -102.0455923789670294, -281.6237833571633473, -301.4846348637937581 ) ) ;
#70021=CARTESIAN_POINT ( 'NONE',  ( -88.45771724803582003, -294.8065940832087790, -327.7034579383222876 ) ) ;
#70022=CARTESIAN_POINT ( 'NONE',  ( 29.64105354140610871, -279.2258184348530676, -234.8427613311651498 ) ) ;
#70023=CARTESIAN_POINT ( 'NONE',  ( -15.56993195612021985, -287.6432004864767578, -196.9624524223594619 ) ) ;
#70024=CARTESIAN_POINT ( 'NONE',  ( 34.75888697250452708, -287.5372221635396386, -281.8646580402398172 ) ) ;
#70026=CARTESIAN_POINT ( 'NONE',  ( -76.71000586960695955, -279.1093007345367027, -332.7175468353536871 ) ) ;
#70027=CARTESIAN_POINT ( 'NONE',  ( -85.55938317218904388, -293.7425687897037392, -327.4105953030698402 ) ) ;
#70028=CARTESIAN_POINT ( 'NONE',  ( -110.3590002741893983, -298.1548430711811193, -282.4626837410476128 ) ) ;
#70029=CARTESIAN_POINT ( 'NONE',  ( -102.2150070530536397, -276.8819810910147226, -304.6916372377997959 ) ) ;
#70032=CARTESIAN_POINT ( 'NONE',  ( -98.21464024813640492, -296.8483285301734895, -223.2205352468766364 ) ) ;
#70033=CARTESIAN_POINT ( 'NONE',  ( -75.43214031300453826, -291.4844407459838180, -334.3325814547297341 ) ) ;
#70034=CARTESIAN_POINT ( 'NONE',  ( 14.94470690833983895, -295.9295690866154018, -325.7919041325711191 ) ) ;
#70037=CARTESIAN_POINT ( 'NONE',  ( -48.06775505554502814, -289.8434933283029977, -342.7229596913379623 ) ) ;
#70040=CARTESIAN_POINT ( 'NONE',  ( 25.73014385346732524, -281.1910097350853448, -314.1422330179764231 ) ) ;
#70041=CARTESIAN_POINT ( 'NONE',  ( -109.3391725997841206, -296.8597198683316947, -297.5238352205884098 ) ) ;
#70042=CARTESIAN_POINT ( 'NONE',  ( -74.05920865460632285, -289.7092062044704903, -204.0879707117975670 ) ) ;
#70043=CARTESIAN_POINT ( 'NONE',  ( 7.969379842708195660, -298.9382089701037444, -193.3797674470473567 ) ) ;
#70048=CARTESIAN_POINT ( 'NONE',  ( -75.30181922533614625, -291.0688199094076367, -336.5558089403842814 ) ) ;
#70049=CARTESIAN_POINT ( 'NONE',  ( -115.3430155898818299, -293.8380690714490129, -288.1317622949166548 ) ) ;
#70051=CARTESIAN_POINT ( 'NONE',  ( 15.09789521561530812, -280.1173063969657733, -214.0441939573391608 ) ) ;
#70052=CARTESIAN_POINT ( 'NONE',  ( -52.48418468218542188, -287.8579096348968278, -197.0758289747388972 ) ) ;
#70053=CARTESIAN_POINT ( 'NONE',  ( 39.01455486600244171, -286.1779079262321375, -274.4099502860120765 ) ) ;
#70054=CARTESIAN_POINT ( 'NONE',  ( -33.93229131641489005, -272.0949882416676928, -195.6054870229756659 ) ) ;
#70055=CARTESIAN_POINT ( 'NONE',  ( -24.36905806254085860, -276.1390528519882537, -197.0075956062217131 ) ) ;
#70056=CARTESIAN_POINT ( 'NONE',  ( -108.3684020862248900, -288.9221122632346237, -248.0354542839610303 ) ) ;
#70057=CARTESIAN_POINT ( 'NONE',  ( -111.2738085925807781, -280.2020354812181040, -286.9245965685014426 ) ) ;
#70060=CARTESIAN_POINT ( 'NONE',  ( -38.35385429679652702, -280.0391191326776834, -197.3557344419517960 ) ) ;
#70061=CARTESIAN_POINT ( 'NONE',  ( 35.23995747301554360, -281.0208500775024731, -279.4791700419551717 ) ) ;
#70062=CARTESIAN_POINT ( 'NONE',  ( -48.43562767465265750, -278.2697369981431166, -346.2990308494979104 ) ) ;
#70063=CARTESIAN_POINT ( 'NONE',  ( -56.44273174643397795, -278.6063596657565427, -196.1231226425536249 ) ) ;
#70064=CARTESIAN_POINT ( 'NONE',  ( 63.33052876804309506, 47.60566335709030739, -316.2373129133302996 ) ) ;
#70065=CARTESIAN_POINT ( 'NONE',  ( -104.0310793156580615, -273.9898844114041481, -232.2366945470407984 ) ) ;
#70066=CARTESIAN_POINT ( 'NONE',  ( -46.08063821706912933, -299.3686419053470331, -194.4517163698844797 ) ) ;
#70068=CARTESIAN_POINT ( 'NONE',  ( -110.4542110544635705, -286.8376638359844719, -287.0812184334320705 ) ) ;
#70071=CARTESIAN_POINT ( 'NONE',  ( 6.038562617998687543, -289.5279785423485919, -329.5207427954307491 ) ) ;
#70072=CARTESIAN_POINT ( 'NONE',  ( 23.34659609950567827, -289.9292637908608299, -316.0875295760779409 ) ) ;
#70073=CARTESIAN_POINT ( 'NONE',  ( -48.08414619837272141, -288.5408766818652566, -342.7205274786652467 ) ) ;
#70074=CARTESIAN_POINT ( 'NONE',  ( -95.29251645813006633, -283.3748125464334748, -320.9697120159855785 ) ) ;
#70075=CARTESIAN_POINT ( 'NONE',  ( -27.43098593705121857, -278.5798868866773432, -197.1778517569633209 ) ) ;
#70076=CARTESIAN_POINT ( 'NONE',  ( -57.75643385455133938, -287.6462839104783029, -198.9346158040809769 ) ) ;
#70077=CARTESIAN_POINT ( 'NONE',  ( 20.71534566357370721, -280.6658037607555798, -315.7493013403125701 ) ) ;
#70078=CARTESIAN_POINT ( 'NONE',  ( -107.7040704593373022, -280.1464140161695582, -249.1389522167001473 ) ) ;
#70079=CARTESIAN_POINT ( 'NONE',  ( -93.64945299741332008, -278.3848553598327271, -316.9363339445436054 ) ) ;
#70080=CARTESIAN_POINT ( 'NONE',  ( -110.4077783357235631, -289.0544869739360365, -293.5422813694628417 ) ) ;
#70081=CARTESIAN_POINT ( 'NONE',  ( -102.3872318523210794, -285.8917376447013226, -229.4558906519198729 ) ) ;
#70082=CARTESIAN_POINT ( 'NONE',  ( -106.6264174583855322, -285.4740623237248087, -236.9073461845415807 ) ) ;
#70083=CARTESIAN_POINT ( 'NONE',  ( 30.33532281853748458, -282.0852809381280508, -297.7257040304157840 ) ) ;
#70086=CARTESIAN_POINT ( 'NONE',  ( -112.1368265475510810, -292.2589893116461326, -282.4439382293692233 ) ) ;
#70088=CARTESIAN_POINT ( 'NONE',  ( -34.95888523483504429, -290.7662912871851972, -193.8783166674654410 ) ) ;
#70089=CARTESIAN_POINT ( 'NONE',  ( 30.39700795093223817, -274.2374291139962565, -242.3913104308159348 ) ) ;
#70091=CARTESIAN_POINT ( 'NONE',  ( -56.05351810221746689, -294.6356332292452294, -344.9478504111654615 ) ) ;
#70092=CARTESIAN_POINT ( 'NONE',  ( -34.81429792446053995, -290.5643519943133697, -196.7111350089235771 ) ) ;
#70093=CARTESIAN_POINT ( 'NONE',  ( -76.20901778210176758, -293.8187902417166129, -333.4074298022957805 ) ) ;
#70094=CONICAL_SURFACE ( 'NONE', #29262, 2.888540232138026020, 0.09862129276974965220 ) ;
#70095=CARTESIAN_POINT ( 'NONE',  ( -76.06527637435584666, -290.7872594468521470, -332.7118609393764359 ) ) ;
#70098=CARTESIAN_POINT ( 'NONE',  ( -110.0618102870256649, -292.7886552846488826, -251.9575803212418350 ) ) ;
#70099=CARTESIAN_POINT ( 'NONE',  ( 37.82368939789227369, -291.5157384831929335, -267.5316428570143330 ) ) ;
#70100=CARTESIAN_POINT ( 'NONE',  ( -47.79790937527012318, -297.1851520823764190, -344.6801606029999334 ) ) ;
#70101=CARTESIAN_POINT ( 'NONE',  ( 7.060094920348323200, -287.6147388181897782, -212.0571258667505106 ) ) ;
#70102=CARTESIAN_POINT ( 'NONE',  ( 31.74191530042645581, -295.9403147691383538, -300.1150034945645189 ) ) ;
#70104=CARTESIAN_POINT ( 'NONE',  ( 0.3503886795678022303, -276.5314665964218079, -205.0950068330576812 ) ) ;
#70106=CARTESIAN_POINT ( 'NONE',  ( -85.10803231170086747, -296.6087331962230564, -210.1736082341220140 ) ) ;
#70107=CARTESIAN_POINT ( 'NONE',  ( 28.92796992001190048, -274.2341822440664600, -303.4357235838158431 ) ) ;
#70108=CARTESIAN_POINT ( 'NONE',  ( -7.398199437998763450, -278.5277091080366745, -202.1951304345557219 ) ) ;
#70109=CARTESIAN_POINT ( 'NONE',  ( -31.32236120155269887, -275.3349129568796343, -197.1985666610361250 ) ) ;
#70110=CARTESIAN_POINT ( 'NONE',  ( 11.42371081850256509, -273.2874553746036099, -211.4659866461770150 ) ) ;
#70113=CARTESIAN_POINT ( 'NONE',  ( -110.8015486704573078, -298.0345106817683245, -265.9992871852042526 ) ) ;
#70115=CARTESIAN_POINT ( 'NONE',  ( -107.0199290459907076, -297.0578817382797183, -292.8307911038286306 ) ) ;
#70117=CARTESIAN_POINT ( 'NONE',  ( -56.88907468414934954, -287.3229788565211607, -343.1907819917381062 ) ) ;
#70118=CARTESIAN_POINT ( 'NONE',  ( -35.81558274971027345, -298.0717807918495623, -197.3611180005151482 ) ) ;
#70120=CARTESIAN_POINT ( 'NONE',  ( 16.29918898183453280, -286.7887501955512448, -215.1193311224510580 ) ) ;
#70121=CARTESIAN_POINT ( 'NONE',  ( -75.65684075173737710, -289.2157159088247340, -337.1270845412653898 ) ) ;
#70122=CARTESIAN_POINT ( 'NONE',  ( -88.51033734342924220, -299.3192809903030707, -214.9715400156740372 ) ) ;
#70123=CARTESIAN_POINT ( 'NONE',  ( -41.15755579295959166, -293.1001064526491291, -345.1099872423227453 ) ) ;
#70124=CARTESIAN_POINT ( 'NONE',  ( 35.17869001448485022, -280.4265417771505895, -244.8062382774861305 ) ) ;
#70125=CARTESIAN_POINT ( 'NONE',  ( -110.4542110544635705, -288.2666405000204577, -253.6410175316879361 ) ) ;
#70126=CARTESIAN_POINT ( 'NONE',  ( -72.05945324018348686, -277.5932229986503330, -203.8239042216753205 ) ) ;
#70129=CARTESIAN_POINT ( 'NONE',  ( -96.88970423976742552, -288.7502650258430208, -313.2699249088517490 ) ) ;
#70131=CARTESIAN_POINT ( 'NONE',  ( -97.38436315569568080, -287.9377561632786069, -315.3256265021667559 ) ) ;
#70132=CARTESIAN_POINT ( 'NONE',  ( -36.49202560124081884, -299.6630912361257515, -196.5608761726103353 ) ) ;
#70133=CARTESIAN_POINT ( 'NONE',  ( 25.45650493751523058, -283.5571519956374686, -313.9156400115997485 ) ) ;
#70134=CARTESIAN_POINT ( 'NONE',  ( -112.7422171607660033, -270.7040298161851410, -264.7091374725872015 ) ) ;
#70135=CARTESIAN_POINT ( 'NONE',  ( 26.45883956513898383, -281.0671197595808621, -234.8858993806427407 ) ) ;
#70136=CARTESIAN_POINT ( 'NONE',  ( -112.3053118441762308, -296.4981134196745529, -288.0095292644644474 ) ) ;
#70137=CARTESIAN_POINT ( 'NONE',  ( -51.69400596789095914, -275.2903632745978939, -198.1328297875758437 ) ) ;
#70138=CARTESIAN_POINT ( 'NONE',  ( 37.19214811362475359, -283.4392933617943413, -261.5587303271289557 ) ) ;
#70139=CARTESIAN_POINT ( 'NONE',  ( -54.26962704452505193, -272.7498925234039007, -199.0332036506258078 ) ) ;
#70141=CARTESIAN_POINT ( 'NONE',  ( 203.9792886337422146, 295.7120653557082619, -54.00000000006011902 ) ) ;
#70142=CARTESIAN_POINT ( 'NONE',  ( -111.0492090421384148, -286.6852204622855993, -258.4880419259926612 ) ) ;
#70145=CARTESIAN_POINT ( 'NONE',  ( -19.05039376806006857, -271.7666405000204009, -190.3683826091709363 ) ) ;
#70146=CARTESIAN_POINT ( 'NONE',  ( -107.4330135628172940, -277.3448988729600160, -301.9766008593547326 ) ) ;
#70147=CARTESIAN_POINT ( 'NONE',  ( -100.0341260492287887, -288.3740368261592835, -313.6750897223426477 ) ) ;
#70148=CARTESIAN_POINT ( 'NONE',  ( -15.91257355089835102, -284.2900160933936036, -340.8699846958140824 ) ) ;
#70149=CARTESIAN_POINT ( 'NONE',  ( 24.45234119004402373, -276.5992226907876557, -230.0134182647407783 ) ) ;
#70150=CARTESIAN_POINT ( 'NONE',  ( -95.80765697662620539, -285.3096222734389471, -319.5782892374174367 ) ) ;
#70151=CARTESIAN_POINT ( 'NONE',  ( -105.5887832998617455, -282.9861027242961882, -297.5081712046438724 ) ) ;
#70152=CARTESIAN_POINT ( 'NONE',  ( -38.40717569289950006, -282.0389554427737835, -195.3559412704315434 ) ) ;
#70153=CARTESIAN_POINT ( 'NONE',  ( -60.87313913315630032, -273.9218203818846860, -196.9892450004276157 ) ) ;
#70154=CARTESIAN_POINT ( 'NONE',  ( 26.93172964526132063, -274.8278898435115707, -227.9591577722697195 ) ) ;
#70155=CARTESIAN_POINT ( 'NONE',  ( -71.57161381736655414, -297.4280830105003588, -336.4785320829901707 ) ) ;
#70159=CARTESIAN_POINT ( 'NONE',  ( -98.08767205084976126, -295.3040801123506753, -225.0599817903433859 ) ) ;
#70160=CARTESIAN_POINT ( 'NONE',  ( 34.22357723811858676, -275.2536962473726021, -285.0716420161719498 ) ) ;
#70162=CARTESIAN_POINT ( 'NONE',  ( -78.05007469219722793, -298.5981637663423953, -205.3663431947522611 ) ) ;
#70163=CARTESIAN_POINT ( 'NONE',  ( 19.42473902992207258, -288.6471739415850379, -222.8487983678375599 ) ) ;
#70164=CARTESIAN_POINT ( 'NONE',  ( -22.21587914087880122, -296.3819188786374639, -345.1536128626588038 ) ) ;
#70165=CARTESIAN_POINT ( 'NONE',  ( 32.95390440070720217, -294.3673171916275351, -239.9220525983916446 ) ) ;
#70166=CARTESIAN_POINT ( 'NONE',  ( -110.9785136476887715, -292.3807953644222266, -283.6895883847779487 ) ) ;
#70167=CARTESIAN_POINT ( 'NONE',  ( 6.005326123405473560, -278.6415284148576461, -209.3605955337199305 ) ) ;
#70169=CARTESIAN_POINT ( 'NONE',  ( -111.7179230733174080, -280.4324571250195959, -273.4419710379085586 ) ) ;
#70170=CARTESIAN_POINT ( 'NONE',  ( -71.61514395911544284, -293.5883958783925323, -336.4559767305045739 ) ) ;
#70171=CARTESIAN_POINT ( 'NONE',  ( -107.0807543817784051, -286.0279732045419223, -300.1055317402342553 ) ) ;
#70172=CARTESIAN_POINT ( 'NONE',  ( -110.4049637105465962, -283.3936745071776500, -276.3599168378987088 ) ) ;
#70173=CARTESIAN_POINT ( 'NONE',  ( 201.4080446206525892, 287.5879394527656814, -97.22726418418297101 ) ) ;
#70175=CARTESIAN_POINT ( 'NONE',  ( -77.05700576180784367, -285.1708569975347132, -209.0248506957818506 ) ) ;
#70177=CARTESIAN_POINT ( 'NONE',  ( 29.49926489302045240, -283.1228378733546833, -308.0696210621243267 ) ) ;
#70179=CARTESIAN_POINT ( 'NONE',  ( -89.26018638665631499, -273.6294670924335151, -219.0136908671740343 ) ) ;
#70180=CARTESIAN_POINT ( 'NONE',  ( 37.90305207048154301, -286.1665472847081446, -256.0001992751724060 ) ) ;
#70182=CARTESIAN_POINT ( 'NONE',  ( 27.64575054332746618, -281.9556242751584136, -229.4026027034914819 ) ) ;
#70183=CARTESIAN_POINT ( 'NONE',  ( -56.72901356050696364, -278.8176855415479736, -344.2183796032391001 ) ) ;
#70184=CARTESIAN_POINT ( 'NONE',  ( 21.88688421964502595, -281.5433865196819170, -221.3173866481988910 ) ) ;
#70185=CARTESIAN_POINT ( 'NONE',  ( -105.5937364680635966, -275.8380690714489560, -285.9065529553535612 ) ) ;
#70186=CARTESIAN_POINT ( 'NONE',  ( -11.98663864091307474, -92.10731666755650338, -360.1219413251452579 ) ) ;
#70188=CARTESIAN_POINT ( 'NONE',  ( 6.223881610526908581, -276.6447947857928966, -209.4524614016336272 ) ) ;
#70189=CARTESIAN_POINT ( 'NONE',  ( 102.4330173972533942, 116.6819059004242121, -282.6453656452667360 ) ) ;
#70191=CARTESIAN_POINT ( 'NONE',  ( -19.10892650690468741, -278.3079144654925585, -197.9238567164312883 ) ) ;
#70192=CARTESIAN_POINT ( 'NONE',  ( 36.09737169397146772, -295.0641840472533204, -250.8000357066200081 ) ) ;
#70193=CARTESIAN_POINT ( 'NONE',  ( -35.65656996429540726, -294.3790745905125164, -343.4561398372795793 ) ) ;
#70194=CARTESIAN_POINT ( 'NONE',  ( -56.16765608581226843, -291.3237198226568694, -195.7065483182462060 ) ) ;
#70196=CARTESIAN_POINT ( 'NONE',  ( -71.82449624844453240, -294.0737123054893800, -338.5486759869114621 ) ) ;
#70197=CARTESIAN_POINT ( 'NONE',  ( 26.37659004006917840, -286.4587747241707802, -307.6967606629390275 ) ) ;
#70198=CARTESIAN_POINT ( 'NONE',  ( 30.98348576775781282, -295.0277830734895588, -241.2032618519249354 ) ) ;
#70199=CARTESIAN_POINT ( 'NONE',  ( -86.06553647444221156, -286.6753809574609022, -215.2728046087326277 ) ) ;
#70201=CARTESIAN_POINT ( 'NONE',  ( -114.1545492466821941, -291.4824016675901248, -271.2380696515119780 ) ) ;
#70202=CARTESIAN_POINT ( 'NONE',  ( 22.63887298028547335, -282.6254565140579871, -312.0782522480375860 ) ) ;
#70203=CARTESIAN_POINT ( 'NONE',  ( -112.8153637342337134, -295.1785656691827171, -283.7659655300626014 ) ) ;
#70204=CIRCLE ( 'NONE', #50584, 5.343514653206204557 ) ;
#70205=CARTESIAN_POINT ( 'NONE',  ( -112.4842181883824708, -291.5569336040776420, -254.2440706921088065 ) ) ;
#70206=CARTESIAN_POINT ( 'NONE',  ( -85.12154886832037448, -290.1837793380809671, -330.7334241161838122 ) ) ;
#70207=CARTESIAN_POINT ( 'NONE',  ( 31.83991718493888712, -287.4093023902037203, -247.0608211935572740 ) ) ;
#70210=CARTESIAN_POINT ( 'NONE',  ( -108.6956664422981476, -298.7393526825194385, -244.8872692269707727 ) ) ;
#70211=CARTESIAN_POINT ( 'NONE',  ( -33.34954539967857556, -296.7859813466320702, -193.8551358194268346 ) ) ;
#70212=CARTESIAN_POINT ( 'NONE',  ( -9.145715563525500968, -279.4888762562534907, -202.7712156085632671 ) ) ;
#70213=CARTESIAN_POINT ( 'NONE',  ( 19.99420486186082613, -274.3627555347478051, -218.9786170727966521 ) ) ;
#70214=CARTESIAN_POINT ( 'NONE',  ( -109.9557685152110196, -295.1962332349838221, -257.7950992953176410 ) ) ;
#70215=CARTESIAN_POINT ( 'NONE',  ( -9.503543598582819385, -278.5449066972386163, -339.1928092203173719 ) ) ;
#70216=CARTESIAN_POINT ( 'NONE',  ( 35.09338491650915870, -273.9032675378040835, -286.6676536452231971 ) ) ;
#70217=CARTESIAN_POINT ( 'NONE',  ( -95.07632328465967930, -297.1216045472151563, -315.6804714105925314 ) ) ;
#70218=CARTESIAN_POINT ( 'NONE',  ( -110.3595161834604284, -297.7248020632274574, -263.2834286698070514 ) ) ;
#70219=CARTESIAN_POINT ( 'NONE',  ( -76.65187845323568183, -297.1687053925359123, -335.6999819723004066 ) ) ;
#70220=CARTESIAN_POINT ( 'NONE',  ( -23.74768633649188843, -296.2217872372291936, -195.1990643542264934 ) ) ;
#70221=CARTESIAN_POINT ( 'NONE',  ( -4.795139363022840051, -293.1438916811865170, -204.8902111711572047 ) ) ;
#70222=CARTESIAN_POINT ( 'NONE',  ( -95.91125400491768005, -274.0270365449062524, -220.6038861598206040 ) ) ;
#70223=CARTESIAN_POINT ( 'NONE',  ( -108.9970896909220954, -289.3469120019418028, -253.5467446630191830 ) ) ;
#70225=CARTESIAN_POINT ( 'NONE',  ( -113.8022095549412853, -273.1516701801307931, -261.7985598755788033 ) ) ;
#70226=CARTESIAN_POINT ( 'NONE',  ( -110.2625633184394331, -296.8349840934420740, -274.1867157484186919 ) ) ;
#70227=CARTESIAN_POINT ( 'NONE',  ( -22.90650122120761267, -282.2157121806354212, -196.3483607646245162 ) ) ;
#70228=CARTESIAN_POINT ( 'NONE',  ( 38.38076764984798217, -280.3745236848430409, -281.2884299263073444 ) ) ;
#70229=CARTESIAN_POINT ( 'NONE',  ( 8.174043579994970443, -275.7967030543647979, -332.4079228316180092 ) ) ;
#70230=CARTESIAN_POINT ( 'NONE',  ( 33.58731567090119086, -279.5936540000705008, -242.3689314604473282 ) ) ;
#70231=CARTESIAN_POINT ( 'NONE',  ( 37.87600967575217226, -279.5469251472152905, -269.9659483041411931 ) ) ;
#70233=CARTESIAN_POINT ( 'NONE',  ( -64.77169839840712484, -272.2615217326580250, -202.0615872460528806 ) ) ;
#70234=CARTESIAN_POINT ( 'NONE',  ( -110.5504780882395153, -280.3423608634501534, -286.7123844378165813 ) ) ;
#70237=CARTESIAN_POINT ( 'NONE',  ( -70.26938460875699377, -295.8640182837222596, -201.8794298262254756 ) ) ;
#70239=CARTESIAN_POINT ( 'NONE',  ( -40.63242019631586999, -292.0118699220529379, -193.4182850485302367 ) ) ;
#70240=CARTESIAN_POINT ( 'NONE',  ( 20.34052322117934963, -278.2166602097238410, -318.5564449296827547 ) ) ;
#70241=CARTESIAN_POINT ( 'NONE',  ( -21.48706350752827987, -272.2552977671797976, -197.0560626092981238 ) ) ;
#70243=CARTESIAN_POINT ( 'NONE',  ( -58.06783165448300821, -285.2378985831060163, -343.0774042051185120 ) ) ;
#70245=CARTESIAN_POINT ( 'NONE',  ( 23.24267728912972686, -284.9485168767567416, -226.0659953627877314 ) ) ;
#70247=CARTESIAN_POINT ( 'NONE',  ( -7.842727875097758705, -293.4517127829731180, -337.5829601827294368 ) ) ;
#70248=CARTESIAN_POINT ( 'NONE',  ( 3.140099106848808663, -284.7418703323610316, -208.1350028090945443 ) ) ;
#70249=CARTESIAN_POINT ( 'NONE',  ( 193.6056169066500274, 279.7126221763799094, -126.0203154767880989 ) ) ;
#70250=CARTESIAN_POINT ( 'NONE',  ( -64.31133829564589632, -293.4037719593771385, -340.3992879172372454 ) ) ;
#70251=CARTESIAN_POINT ( 'NONE',  ( 7.155476341450177635, -285.1256556595370739, -208.3064391421114578 ) ) ;
#70252=CARTESIAN_POINT ( 'NONE',  ( -27.47133515261248249, -281.7796282053889172, -197.1723980869047637 ) ) ;
#70253=CARTESIAN_POINT ( 'NONE',  ( -10.14934143917211884, -287.6042921766826339, -198.6904798207445992 ) ) ;
#70254=CARTESIAN_POINT ( 'NONE',  ( 30.16648155789390273, -280.2476415581548395, -305.2411898978089084 ) ) ;
#70255=CARTESIAN_POINT ( 'NONE',  ( 23.50949717981876219, -288.1119817840691439, -310.7092745384828163 ) ) ;
#70257=CARTESIAN_POINT ( 'NONE',  ( -37.02385347869132914, -281.4814833932616693, -196.7725734079370454 ) ) ;
#70258=CARTESIAN_POINT ( 'NONE',  ( -39.71669486285533424, -280.8244339688591253, -197.2256526752249499 ) ) ;
#70259=CARTESIAN_POINT ( 'NONE',  ( -15.90600449527480897, -288.3078116544500631, -198.0648377633520170 ) ) ;
#70261=CARTESIAN_POINT ( 'NONE',  ( -54.59310246451565263, -297.6696818863487692, -195.3185359247007682 ) ) ;
#70262=CARTESIAN_POINT ( 'NONE',  ( -93.81709411303738477, -293.2121608428080322, -221.5515218024827675 ) ) ;
#70264=CARTESIAN_POINT ( 'NONE',  ( 108.5619616845123971, -302.2645883696979467, -190.3030568020281805 ) ) ;
#70266=CARTESIAN_POINT ( 'NONE',  ( 0.2999342423192604135, -272.5520562232745760, -205.2836413248113843 ) ) ;
#70268=CARTESIAN_POINT ( 'NONE',  ( -74.23705991405583404, -293.9336245985008418, -337.0923468979850668 ) ) ;
#70269=CARTESIAN_POINT ( 'NONE',  ( -84.10942055557747210, -296.8968344065521023, -214.1633592599051781 ) ) ;
#70270=CARTESIAN_POINT ( 'NONE',  ( -58.87339304845819044, -290.8557890698519373, -340.8920315504221321 ) ) ;
#70272=CARTESIAN_POINT ( 'NONE',  ( 24.51730149701409545, -282.7554761154105449, -229.6308450041551055 ) ) ;
#70273=CARTESIAN_POINT ( 'NONE',  ( -62.55198748662395047, -290.7990188331613695, -342.5492201428829731 ) ) ;
#70274=CARTESIAN_POINT ( 'NONE',  ( -112.6449147126792383, -291.6962458976706785, -283.9525761666745325 ) ) ;
#70275=CARTESIAN_POINT ( 'NONE',  ( -91.11408915279824328, -287.2888084187766822, -218.0033848817627131 ) ) ;
#70276=CARTESIAN_POINT ( 'NONE',  ( 10.82135480106749092, -280.8636275364432890, -210.2151607901950285 ) ) ;
#70277=CARTESIAN_POINT ( 'NONE',  ( -110.8673717908075247, -294.8539699541096866, -252.9459002434879551 ) ) ;
#70278=CARTESIAN_POINT ( 'NONE',  ( -35.90132357153543552, -282.8679097882399560, -347.3607618358029754 ) ) ;
#70279=CARTESIAN_POINT ( 'NONE',  ( 35.37926986804953344, -277.6060787597874082, -285.2784235686195871 ) ) ;
#70280=CARTESIAN_POINT ( 'NONE',  ( -67.74223827176244583, -276.1233781216987495, -207.3071070584150277 ) ) ;
#70281=CARTESIAN_POINT ( 'NONE',  ( 18.14770556826152159, -274.5095428760557184, -322.2735429811021390 ) ) ;
#70283=CARTESIAN_POINT ( 'NONE',  ( 23.73742078915519826, -280.5033509488308141, -230.1783568695826148 ) ) ;
#70284=CARTESIAN_POINT ( 'NONE',  ( -84.60924697647813275, -278.8916447344553262, -330.7094156097239193 ) ) ;
#70285=CARTESIAN_POINT ( 'NONE',  ( -109.7513235723459246, -283.9334340416561417, -244.8725588767660213 ) ) ;
#70286=CARTESIAN_POINT ( 'NONE',  ( 2.771125923696083682, -294.3581215681567187, -208.0996517589562416 ) ) ;
#70287=CARTESIAN_POINT ( 'NONE',  ( -76.04415078586332299, -275.1447050386446449, -204.6605124888353373 ) ) ;
#70289=CARTESIAN_POINT ( 'NONE',  ( -34.14069766185071586, -275.4067897676488315, -193.9212602059480162 ) ) ;
#70291=CARTESIAN_POINT ( 'NONE',  ( 35.35381607985218722, -275.4733338648393897, -277.0215930222729526 ) ) ;
#70293=CARTESIAN_POINT ( 'NONE',  ( -110.5785107945265509, -298.7509451813999135, -254.9241625969769132 ) ) ;
#70294=CARTESIAN_POINT ( 'NONE',  ( -110.4506616161603318, -282.7582995415833125, -254.3292779525702088 ) ) ;
#70295=CARTESIAN_POINT ( 'NONE',  ( -37.79064699900006730, -291.7133938579762003, -193.3835710070106018 ) ) ;
#70296=CARTESIAN_POINT ( 'NONE',  ( 35.11164791481240854, -273.3405586240686489, -252.4067546239757576 ) ) ;
#70297=CARTESIAN_POINT ( 'NONE',  ( 35.62529218920555252, -289.4313103761550678, -292.3668612921380827 ) ) ;
#70298=CARTESIAN_POINT ( 'NONE',  ( -99.96857200631606588, -289.9950998411681553, -232.2546750636778654 ) ) ;
#70299=ORIENTED_EDGE ( 'NONE', *, *, #85455, .F. ) ;
#70300=CARTESIAN_POINT ( 'NONE',  ( -47.64582717111662902, -290.4984690050655445, -194.5949154214187047 ) ) ;
#70301=CARTESIAN_POINT ( 'NONE',  ( -79.53946562107320517, -291.1314442144685586, -210.7052165904021592 ) ) ;
#70303=CARTESIAN_POINT ( 'NONE',  ( 25.60589750796334130, -289.2140786410971032, -314.2597679163053499 ) ) ;
#70304=CARTESIAN_POINT ( 'NONE',  ( -70.95517775584033870, -279.9291345889272975, -205.5224812524338631 ) ) ;
#70305=CARTESIAN_POINT ( 'NONE',  ( -0.8653597404803231585, -293.4997981559777713, -337.8368132333877156 ) ) ;
#70306=CARTESIAN_POINT ( 'NONE',  ( -7.390497174086534393, -287.0860008576058249, -199.4791340293585904 ) ) ;
#70307=CARTESIAN_POINT ( 'NONE',  ( -114.3056797163455229, -284.9259843041483009, -267.1195321435994856 ) ) ;
#70308=CARTESIAN_POINT ( 'NONE',  ( 35.72403600755610142, -281.8979466298940793, -271.3097986877388053 ) ) ;
#70309=CARTESIAN_POINT ( 'NONE',  ( -107.8472915499240230, -262.5275434182412937, -317.6634998498594200 ) ) ;
#70310=CARTESIAN_POINT ( 'NONE',  ( 83.29146807913110706, 83.53839643160537776, -301.3178837860347130 ) ) ;
#70311=CARTESIAN_POINT ( 'NONE',  ( 187.7931042187957189, 269.0293024058671563, -137.6635259067655568 ) ) ;
#70312=CARTESIAN_POINT ( 'NONE',  ( 34.53404840778943452, -274.5695729566004957, -256.7054049009872756 ) ) ;
#70313=CARTESIAN_POINT ( 'NONE',  ( 1.021519072595784339, -275.4477503498168858, -332.8906680306652106 ) ) ;
#70314=CARTESIAN_POINT ( 'NONE',  ( -114.2479071756398525, -296.1052303320313399, -266.7319245010062900 ) ) ;
#70315=CARTESIAN_POINT ( 'NONE',  ( -109.2583768833345346, -269.3191087492390920, -295.4032835330162357 ) ) ;
#70316=CARTESIAN_POINT ( 'NONE',  ( 37.42017352094932647, -274.4422531652433008, -286.6691281790893413 ) ) ;
#70317=CARTESIAN_POINT ( 'NONE',  ( -74.80539363038832334, -275.3066419526037407, -206.4703545262239572 ) ) ;
#70319=CARTESIAN_POINT ( 'NONE',  ( -112.3730818592268861, -297.6976051538242132, -254.0789924899772814 ) ) ;
#70320=CARTESIAN_POINT ( 'NONE',  ( 10.16002664193914917, -288.8688850165066810, -325.9399473659889850 ) ) ;
#70321=CARTESIAN_POINT ( 'NONE',  ( -93.56433119474081650, -296.6393211319078773, -322.7558176957816158 ) ) ;
#70322=CARTESIAN_POINT ( 'NONE',  ( -93.64016104097697735, -296.3288858487308630, -322.8210595970627992 ) ) ;
#70323=CARTESIAN_POINT ( 'NONE',  ( 28.73761629076754787, -293.2983231851065398, -239.2172540221910140 ) ) ;
#70324=ORIENTED_EDGE ( 'NONE', *, *, #43435, .F. ) ;
#70325=AXIS2_PLACEMENT_3D ( 'NONE', #86639, #58717, #80943 ) ;
#70326=CARTESIAN_POINT ( 'NONE',  ( 31.71382831265789193, -277.8711922514915500, -301.0311063593334211 ) ) ;
#70327=ORIENTED_EDGE ( 'NONE', *, *, #14172, .F. ) ;
#70328=CARTESIAN_POINT ( 'NONE',  ( -33.91173708077440807, -279.6018746095932670, -193.4991491237396417 ) ) ;
#70330=CARTESIAN_POINT ( 'NONE',  ( -43.21404479819425859, -278.0693793825921603, -343.3605975443823013 ) ) ;
#70331=CARTESIAN_POINT ( 'NONE',  ( 0.6688505955550543280, -276.3117510966048371, -204.5495922861765621 ) ) ;
#70332=CARTESIAN_POINT ( 'NONE',  ( -76.97180381096681856, -275.5999126088041749, -334.5143685359605570 ) ) ;
#70333=CARTESIAN_POINT ( 'NONE',  ( -91.92652286646358561, -297.8979031564689990, -221.7361265174787093 ) ) ;
#70335=CARTESIAN_POINT ( 'NONE',  ( -99.23866911703809990, -294.5793800156246220, -310.2557597311214863 ) ) ;
#70337=CARTESIAN_POINT ( 'NONE',  ( 35.26752485054985442, -281.7215128284715320, -244.7574394713518302 ) ) ;
#70338=CARTESIAN_POINT ( 'NONE',  ( 29.15513977667851009, -276.1247760911959404, -300.4803856888670452 ) ) ;
#70340=CARTESIAN_POINT ( 'NONE',  ( 25.95881791097069424, -285.6665569705854750, -227.3686180763505149 ) ) ;
#70341=CARTESIAN_POINT ( 'NONE',  ( -103.8475580135583556, -275.0127505345258783, -235.5793378281366870 ) ) ;
#70343=CARTESIAN_POINT ( 'NONE',  ( 33.85587433152726788, -286.9709573917939451, -287.1987876137876583 ) ) ;
#70344=CARTESIAN_POINT ( 'NONE',  ( -8.836647185372752844, -278.6701192954755584, -202.0571212369497971 ) ) ;
#70345=CARTESIAN_POINT ( 'NONE',  ( -67.53155515161816425, -278.2228937145070518, -203.2359474512934128 ) ) ;
#70346=CARTESIAN_POINT ( 'NONE',  ( -79.20627427203412196, -281.7018087495495138, -331.9133041952593999 ) ) ;
#70347=CARTESIAN_POINT ( 'NONE',  ( 29.07781926739929190, -289.0895138703878047, -235.4160744100857983 ) ) ;
#70348=CARTESIAN_POINT ( 'NONE',  ( 14.02009782656586268, -277.5170055668595523, -322.8637408111001719 ) ) ;
#70350=CARTESIAN_POINT ( 'NONE',  ( -89.41610783252477290, -293.3193760031869033, -216.3144224936077364 ) ) ;
#70351=CARTESIAN_POINT ( 'NONE',  ( -39.95090737751955601, -275.3243437782816727, -346.3158716445261689 ) ) ;
#70352=CARTESIAN_POINT ( 'NONE',  ( 31.36040426466440323, -276.5376682192219278, -295.4865229812849634 ) ) ;
#70353=CARTESIAN_POINT ( 'NONE',  ( 1.177063809260052718, -284.5392268197408043, -334.9082577420206803 ) ) ;
#70355=CARTESIAN_POINT ( 'NONE',  ( -112.3804373308198592, -292.3538969915509824, -279.6519411409492477 ) ) ;
#70356=CARTESIAN_POINT ( 'NONE',  ( -109.7278565081622475, -294.8049147501040466, -250.6854236694423435 ) ) ;
#70357=CARTESIAN_POINT ( 'NONE',  ( -85.40393358707706284, -284.6039895329334399, -210.4096331391698982 ) ) ;
#70358=CARTESIAN_POINT ( 'NONE',  ( 120.8395553409046528, -299.5541904835127980, -193.1741385666954898 ) ) ;
#70359=CARTESIAN_POINT ( 'NONE',  ( 0.8831657230102820666, -273.2586099572882290, -207.5908773543315817 ) ) ;
#70360=CARTESIAN_POINT ( 'NONE',  ( 0.5597263908309599856, -290.7027243267227732, -206.5305034773938928 ) ) ;
#70363=CARTESIAN_POINT ( 'NONE',  ( -109.7666508136769750, -289.3391132043227572, -246.1681118314136256 ) ) ;
#70364=CARTESIAN_POINT ( 'NONE',  ( -99.69617312076667304, -285.6115192369749707, -309.9328171761367798 ) ) ;
#70365=CARTESIAN_POINT ( 'NONE',  ( -7.717229398908735938, -284.6748359554690069, -200.3311702558887646 ) ) ;
#70366=CARTESIAN_POINT ( 'NONE',  ( -94.59180408132135653, -286.6262451252516712, -224.1047848647469323 ) ) ;
#70367=CARTESIAN_POINT ( 'NONE',  ( -8.200002786311845426, -287.2466821978695179, -203.2540155016641279 ) ) ;
#70368=CARTESIAN_POINT ( 'NONE',  ( -30.86433191212338656, -294.1133918285856907, -195.2331887625418858 ) ) ;
#70369=CARTESIAN_POINT ( 'NONE',  ( -15.03852053104803943, -274.8454834371672746, -342.6092616765690764 ) ) ;
#70370=CARTESIAN_POINT ( 'NONE',  ( 38.70605821425171200, -275.7350446589559283, -258.3395677487113744 ) ) ;
#70371=CARTESIAN_POINT ( 'NONE',  ( 12.35019880327456399, -290.8176870250891284, -213.4398620582861668 ) ) ;
#70372=CARTESIAN_POINT ( 'NONE',  ( -108.6564331676212447, -278.1833601874256487, -299.3991766556042649 ) ) ;
#70373=CARTESIAN_POINT ( 'NONE',  ( -36.96242811806868644, -297.0272377422477916, -345.0176632965091699 ) ) ;
#70376=CARTESIAN_POINT ( 'NONE',  ( -87.27610497077372997, -282.4502683532564333, -324.3547651650628154 ) ) ;
#70377=CARTESIAN_POINT ( 'NONE',  ( -106.6543584422696824, -276.9258367037618314, -241.7122778040967432 ) ) ;
#70379=CARTESIAN_POINT ( 'NONE',  ( -34.11298181892665582, -272.5719519753736222, -194.1227868622081871 ) ) ;
#70380=CARTESIAN_POINT ( 'NONE',  ( -91.04836999871002945, -277.1887992585210441, -320.0279663859444099 ) ) ;
#70381=CARTESIAN_POINT ( 'NONE',  ( -0.3937189787852397593, -296.0719105576415018, -334.1810671305825053 ) ) ;
#70382=CARTESIAN_POINT ( 'NONE',  ( 36.69023775462581227, -280.2202080807005018, -250.2921754138708934 ) ) ;
#70383=CARTESIAN_POINT ( 'NONE',  ( -6.655435022424898150, -295.5803027959955216, -336.8574455707059769 ) ) ;
#70384=CARTESIAN_POINT ( 'NONE',  ( -50.36697883633235762, -296.5301414763106891, -345.8046382676407120 ) ) ;
#70385=CARTESIAN_POINT ( 'NONE',  ( 51.67140180705295904, -299.0303371588389041, -197.3637701282314367 ) ) ;
#70386=CARTESIAN_POINT ( 'NONE',  ( -89.33494695934896868, -293.3208142704036732, -216.2365416088703682 ) ) ;
#70387=CARTESIAN_POINT ( 'NONE',  ( -18.18407961466337142, -286.4590021806242817, -195.7272952184086989 ) ) ;
#70388=CARTESIAN_POINT ( 'NONE',  ( 38.39673295420836041, -273.6663299575354245, -268.3623103142480204 ) ) ;
#70389=CARTESIAN_POINT ( 'NONE',  ( -28.97928851788870475, -288.7823927679049234, -346.9592064938008207 ) ) ;
#70390=CARTESIAN_POINT ( 'NONE',  ( -107.0593680910357648, -280.8820552013037855, -243.5461288344261561 ) ) ;
#70391=CARTESIAN_POINT ( 'NONE',  ( -101.1906023740660743, -284.1013890589640596, -234.3862549440055147 ) ) ;
#70392=CARTESIAN_POINT ( 'NONE',  ( -110.3640301712797509, -288.7716880691907591, -253.2514725013641623 ) ) ;
#70393=CARTESIAN_POINT ( 'NONE',  ( -107.5887910744927609, -275.4946769126667618, -270.3985833712262092 ) ) ;
#70394=CARTESIAN_POINT ( 'NONE',  ( 23.58884919973117889, -286.4998199235967036, -229.9525588811646060 ) ) ;
#70396=CARTESIAN_POINT ( 'NONE',  ( 22.34789876270433240, -283.1428196582348278, -318.6516454077776643 ) ) ;
#70397=CARTESIAN_POINT ( 'NONE',  ( -86.35356385484118391, -290.4499913419300583, -211.2103214523775137 ) ) ;
#70398=CARTESIAN_POINT ( 'NONE',  ( -94.37667358441451881, -280.8440455433234320, -219.8294227883827716 ) ) ;
#70400=CARTESIAN_POINT ( 'NONE',  ( -112.2382481018925802, -280.0646488581643325, -254.6836037667670780 ) ) ;
#70401=CARTESIAN_POINT ( 'NONE',  ( 21.33024004803469964, -280.7762299713866696, -226.9050300157267372 ) ) ;
#70402=CARTESIAN_POINT ( 'NONE',  ( 32.01487516473824968, -277.1783681150890288, -241.6825061669991612 ) ) ;
#70403=CARTESIAN_POINT ( 'NONE',  ( 23.17167253478684330, -294.1891097677450944, -317.9966791641726331 ) ) ;
#70404=CARTESIAN_POINT ( 'NONE',  ( -109.9562191162959124, -288.3491720125779239, -287.6521109819722710 ) ) ;
#70406=CARTESIAN_POINT ( 'NONE',  ( -82.12211458236384942, -296.3456210552271841, -212.2542148528756911 ) ) ;
#70409=CARTESIAN_POINT ( 'NONE',  ( -2.934474104838156627, -284.5139946081728795, -336.3864382472799548 ) ) ;
#70410=CARTESIAN_POINT ( 'NONE',  ( -75.67276744759786311, -295.2454202719474665, -332.5716325998578213 ) ) ;
#70411=CARTESIAN_POINT ( 'NONE',  ( 22.85684462535671102, -293.9935047048724073, -222.8256381593327546 ) ) ;
#70412=CARTESIAN_POINT ( 'NONE',  ( -10.93121159424621780, -283.3500625993008839, -338.5791273654646147 ) ) ;
#70413=CARTESIAN_POINT ( 'NONE',  ( 32.34451463327189913, -274.1962932348337745, -238.0374159404958334 ) ) ;
#70414=CARTESIAN_POINT ( 'NONE',  ( -112.4639845129818951, -290.9978056478661870, -286.7914306978094032 ) ) ;
#70415=CARTESIAN_POINT ( 'NONE',  ( -67.97920228707845069, -283.7938315207817936, -201.0530431313786721 ) ) ;
#70416=CARTESIAN_POINT ( 'NONE',  ( -111.9751168400454446, -291.1220455917654704, -251.4507212874577817 ) ) ;
#70417=CARTESIAN_POINT ( 'NONE',  ( 33.04851782932698256, -287.6288386330920730, -250.9367852337041143 ) ) ;
#70420=CARTESIAN_POINT ( 'NONE',  ( 173.3795401471607249, 240.5383949446079441, -177.0376500821581089 ) ) ;
#70421=CARTESIAN_POINT ( 'NONE',  ( -81.14755544000014709, -285.1552235838548199, -332.9054245497384272 ) ) ;
#70422=CARTESIAN_POINT ( 'NONE',  ( 21.31550574532286291, -290.4094976428776249, -223.6242672951989618 ) ) ;
#70424=CARTESIAN_POINT ( 'NONE',  ( 20.76934989462517933, -279.8459479456881809, -225.6491903601987872 ) ) ;
#70425=CARTESIAN_POINT ( 'NONE',  ( 35.17962102336328911, -275.5465393844146433, -296.3329793798410492 ) ) ;
#70426=CARTESIAN_POINT ( 'NONE',  ( -107.9866991209911475, -280.2301735140410983, -295.2023742165029034 ) ) ;
#70427=CARTESIAN_POINT ( 'NONE',  ( -20.06228311212446158, -109.6411408614775098, -360.8968400945585131 ) ) ;
#70428=CARTESIAN_POINT ( 'NONE',  ( 26.22158160618183231, -280.6893963199886457, -312.7676682769504737 ) ) ;
#70429=CARTESIAN_POINT ( 'NONE',  ( -90.82413384932404199, -283.3093974308474685, -218.2151351854687391 ) ) ;
#70430=CARTESIAN_POINT ( 'NONE',  ( -112.7716210525488094, -298.4286507919750306, -261.1795580784037156 ) ) ;
#70431=CARTESIAN_POINT ( 'NONE',  ( 12.94097172995459211, -293.2699203188096249, -217.3550678338742443 ) ) ;
#70433=CARTESIAN_POINT ( 'NONE',  ( -109.6671955743595817, -289.0659965806693208, -283.4097266189107813 ) ) ;
#70434=CARTESIAN_POINT ( 'NONE',  ( -45.63037386966995257, -277.8058605918876651, -346.8641594955472556 ) ) ;
#70435=CARTESIAN_POINT ( 'NONE',  ( -36.48553719244878124, -298.2298444201506413, -197.3610928647055971 ) ) ;
#70437=CARTESIAN_POINT ( 'NONE',  ( -93.90793867459910871, -272.1798830500507620, -218.5560862486163387 ) ) ;
#70440=CARTESIAN_POINT ( 'NONE',  ( 33.95398569155008772, -282.8566693598043003, -287.4777196629380001 ) ) ;
#70441=CARTESIAN_POINT ( 'NONE',  ( 5.592988562297290578, -282.3851735003717636, -207.6667281306568213 ) ) ;
#70442=CARTESIAN_POINT ( 'NONE',  ( -100.6104141097120248, -283.1063119040639435, -307.2457798186815126 ) ) ;
#70443=CARTESIAN_POINT ( 'NONE',  ( -37.02646435070128206, -281.9165565869342345, -196.1265834965426791 ) ) ;
#70444=CARTESIAN_POINT ( 'NONE',  ( 34.51409877170166141, -273.8176575088681375, -253.9506748952433099 ) ) ;
#70447=CARTESIAN_POINT ( 'NONE',  ( -72.75714463488614570, -278.3119017690627857, -338.5660027969175303 ) ) ;
#70451=CARTESIAN_POINT ( 'NONE',  ( -113.0926791583531781, -286.4528732810155134, -267.1901203344636997 ) ) ;
#70452=CARTESIAN_POINT ( 'NONE',  ( 35.58457702316624705, -292.8264702047973174, -276.2228436234940432 ) ) ;
#70453=CARTESIAN_POINT ( 'NONE',  ( 10.15845928634537820, -287.7655187065291784, -330.9023823249069096 ) ) ;
#70454=CARTESIAN_POINT ( 'NONE',  ( -41.35578234679477561, -284.2408107500264123, -196.4440404413563499 ) ) ;
#70455=CARTESIAN_POINT ( 'NONE',  ( -108.9345668287926401, -283.3503187269599835, -253.2823250766483909 ) ) ;
#70456=CARTESIAN_POINT ( 'NONE',  ( -71.66228721505896715, -287.7519132252717213, -335.9503674799708506 ) ) ;
#70457=CARTESIAN_POINT ( 'NONE',  ( -96.23120351448213228, -285.1460434797748462, -314.1693009701115784 ) ) ;
#70458=CARTESIAN_POINT ( 'NONE',  ( 18.37392987649216991, -274.2519160757052532, -320.5875924219042190 ) ) ;
#70459=CARTESIAN_POINT ( 'NONE',  ( -33.74449561457781499, -284.4965878972702171, -194.2460699548436480 ) ) ;
#70460=CARTESIAN_POINT ( 'NONE',  ( -36.59203453992425636, -300.0616930923462178, -195.3608536800668105 ) ) ;
#70461=CARTESIAN_POINT ( 'NONE',  ( -66.45489673066794012, -283.6716376144769924, -201.0614050545398186 ) ) ;
#70462=CARTESIAN_POINT ( 'NONE',  ( 32.95709836510569346, -282.2226865089769490, -249.8309601934315936 ) ) ;
#70463=CARTESIAN_POINT ( 'NONE',  ( 36.86922392046123065, -289.7094520682850316, -282.6267391372953171 ) ) ;
#70465=CARTESIAN_POINT ( 'NONE',  ( -2.607253171737097919, -296.5165584644005889, -337.4642654165792806 ) ) ;
#70466=CARTESIAN_POINT ( 'NONE',  ( -34.20486192780585100, -278.0914102157768752, -195.4138537235818376 ) ) ;
#70467=CARTESIAN_POINT ( 'NONE',  ( -104.4639435055522085, -290.2352048047389985, -232.9610743457317028 ) ) ;
#70468=CARTESIAN_POINT ( 'NONE',  ( -66.38654922876303033, -293.8388077363383672, -338.2053303899429011 ) ) ;
#70469=CARTESIAN_POINT ( 'NONE',  ( -107.6943845293313871, -277.5164906040081974, -249.1068648560783743 ) ) ;
#70470=CARTESIAN_POINT ( 'NONE',  ( -39.17548730034383198, -296.1685143501420043, -196.1359479003110096 ) ) ;
#70471=CARTESIAN_POINT ( 'NONE',  ( 35.78425105212308921, -294.7647574848086265, -262.5328525572728040 ) ) ;
#70472=CARTESIAN_POINT ( 'NONE',  ( 35.78497577281001440, -290.2662352645559167, -287.0191576251351080 ) ) ;
#70473=CARTESIAN_POINT ( 'NONE',  ( -113.6444734326017283, -295.0417619637821076, -269.5900557760484730 ) ) ;
#70474=CARTESIAN_POINT ( 'NONE',  ( 4.080296576367366868, -290.0842725910494551, -331.5018673095632948 ) ) ;
#70475=CARTESIAN_POINT ( 'NONE',  ( 33.52598945148352527, -291.4383954758265531, -242.7976370683088874 ) ) ;
#70476=CARTESIAN_POINT ( 'NONE',  ( -105.2537969564822333, -292.3561414895329449, -241.8854979274368588 ) ) ;
#70478=CARTESIAN_POINT ( 'NONE',  ( -70.30260065243886913, -292.4089624490845836, -205.0451110309617491 ) ) ;
#70480=CARTESIAN_POINT ( 'NONE',  ( -110.0588545373884273, -292.0638715102076617, -246.1071754726964116 ) ) ;
#70481=CARTESIAN_POINT ( 'NONE',  ( 16.63022849512995194, -280.3097522843655725, -323.0230798578372742 ) ) ;
#70482=CARTESIAN_POINT ( 'NONE',  ( 35.42443431690416134, -293.6291734838542311, -276.1997546328657904 ) ) ;
#70483=CARTESIAN_POINT ( 'NONE',  ( 39.64064422321507664, -281.5108343277557879, -267.0573769879011365 ) ) ;
#70484=CARTESIAN_POINT ( 'NONE',  ( -105.7672995175042701, -283.7629100493165311, -305.7433051657801002 ) ) ;
#70485=CARTESIAN_POINT ( 'NONE',  ( -34.53410916004471432, -287.0167631654152842, -345.1925978278831622 ) ) ;
#70486=CARTESIAN_POINT ( 'NONE',  ( -74.43418150951416123, -281.6902171684786254, -334.7237745564837041 ) ) ;
#70487=CARTESIAN_POINT ( 'NONE',  ( -88.50284191313016890, -283.3351405266946017, -215.4494796820675901 ) ) ;
#70489=CARTESIAN_POINT ( 'NONE',  ( -11.72372324553491829, -278.8595073497788803, -198.4277721252866797 ) ) ;
#70490=CARTESIAN_POINT ( 'NONE',  ( 2.591835866407439237, -285.4947844899659799, -204.8874193511742590 ) ) ;
#70492=CARTESIAN_POINT ( 'NONE',  ( -14.61923420005219754, -293.9517609463957797, -200.1462338332117383 ) ) ;
#70493=CARTESIAN_POINT ( 'NONE',  ( 0.8848012538291770701, -275.9769362108248174, -204.1844758618515527 ) ) ;
#70494=CARTESIAN_POINT ( 'NONE',  ( -105.2890244228423740, -277.8613220640744430, -297.1052501967619150 ) ) ;
#70495=CARTESIAN_POINT ( 'NONE',  ( -64.39079182615223829, -291.8755264076513640, -198.2123187016681527 ) ) ;
#70496=CARTESIAN_POINT ( 'NONE',  ( -63.43805831982277255, -281.4694368201828070, -341.2715846753409892 ) ) ;
#70497=EDGE_CURVE ( 'NONE', #64642, #9910, #68518, .T. ) ;
#70498=CARTESIAN_POINT ( 'NONE',  ( -34.83726953145153260, -291.1431283816995688, -197.1686574687067264 ) ) ;
#70499=CARTESIAN_POINT ( 'NONE',  ( -90.20725363860721302, -295.3043287389435250, -217.1611753172365127 ) ) ;
#70502=CARTESIAN_POINT ( 'NONE',  ( 14.92391109133455984, -292.3211182338945946, -219.2367707040171467 ) ) ;
#70504=CARTESIAN_POINT ( 'NONE',  ( -102.0455923789670294, -275.6237833571633473, -301.4846348637937581 ) ) ;
#70505=CARTESIAN_POINT ( 'NONE',  ( -96.33830285497202794, -294.9480838607117335, -319.4959286018274724 ) ) ;
#70506=CARTESIAN_POINT ( 'NONE',  ( -9.295961007020183686, -278.5544922487031840, -199.9782933864558458 ) ) ;
#70507=CARTESIAN_POINT ( 'NONE',  ( -102.1099567258476810, -286.4039964930817632, -229.6380138591213438 ) ) ;
#70508=CARTESIAN_POINT ( 'NONE',  ( 4.727098966536575020, -286.4710138708360319, -210.6400924584868619 ) ) ;
#70509=CARTESIAN_POINT ( 'NONE',  ( -4.742113838513839497, -278.1349480867809234, -336.4657971616366581 ) ) ;
#70510=CARTESIAN_POINT ( 'NONE',  ( -83.39395379547509890, -293.7065546999000958, -329.1725608119978119 ) ) ;
#70511=CARTESIAN_POINT ( 'NONE',  ( -91.12843962527867347, -297.5892523712590219, -321.2774091184696204 ) ) ;
#70512=CARTESIAN_POINT ( 'NONE',  ( -91.26997362820775095, -276.6352260836397932, -320.2233339681659459 ) ) ;
#70515=CARTESIAN_POINT ( 'NONE',  ( -90.70047796957018704, -295.4502669847406082, -325.9195091387227876 ) ) ;
#70516=CARTESIAN_POINT ( 'NONE',  ( -71.81839302994913510, -291.4316134962004980, -336.3502989366946849 ) ) ;
#70519=CARTESIAN_POINT ( 'NONE',  ( 16.09113264438434854, -288.9207513429436744, -320.3233196171364625 ) ) ;
#70521=CARTESIAN_POINT ( 'NONE',  ( -39.56838718495048113, -279.0836178488788164, -193.6157013656127504 ) ) ;
#70522=CARTESIAN_POINT ( 'NONE',  ( -98.18870956582244958, -296.5750772831426048, -317.3819030626211770 ) ) ;
#70523=CARTESIAN_POINT ( 'NONE',  ( -111.9514636064411093, -288.8592497763979168, -257.1820180260689881 ) ) ;
#70524=CARTESIAN_POINT ( 'NONE',  ( -99.90684308770038058, -297.4798921422525382, -225.5130725624387082 ) ) ;
#70525=CARTESIAN_POINT ( 'NONE',  ( 28.41543976323979592, -294.3163836630541255, -302.2281114412960505 ) ) ;
#70529=CARTESIAN_POINT ( 'NONE',  ( 26.87191746113027335, -289.6190549378038668, -311.6813801045261130 ) ) ;
#70530=CARTESIAN_POINT ( 'NONE',  ( 40.64545035920995986, -277.8376638359844719, -252.5284128619064461 ) ) ;
#70532=CARTESIAN_POINT ( 'NONE',  ( 36.50415773423206645, -280.6308635198334400, -248.8639039775103754 ) ) ;
#70533=CARTESIAN_POINT ( 'NONE',  ( -111.3065374100586382, -286.4017563320265936, -282.0608388809010876 ) ) ;
#70534=CARTESIAN_POINT ( 'NONE',  ( 7.215181859690259714, -285.2204900623581807, -208.2210605758807276 ) ) ;
#70535=CARTESIAN_POINT ( 'NONE',  ( -91.50643881267039603, -271.2786216153082250, -218.7070261488613028 ) ) ;
#70536=CARTESIAN_POINT ( 'NONE',  ( -109.7568286238355455, -288.4089004734184414, -287.6053450330914529 ) ) ;
#70537=CARTESIAN_POINT ( 'NONE',  ( 28.04214118035680769, -277.9189128043040000, -308.6398166849419908 ) ) ;
#70539=CARTESIAN_POINT ( 'NONE',  ( -95.27301981713750934, -277.9272385251546211, -314.7791571005171249 ) ) ;
#70540=CARTESIAN_POINT ( 'NONE',  ( -35.65213787455041228, -279.4224568114539125, -197.2662921318444376 ) ) ;
#70541=CARTESIAN_POINT ( 'NONE',  ( 5.709167299155815556, -277.5632098443919062, -333.8285531193897668 ) ) ;
#70542=CARTESIAN_POINT ( 'NONE',  ( -112.1002724823039216, -277.1370401253649902, -287.0693369216727433 ) ) ;
#70543=CARTESIAN_POINT ( 'NONE',  ( -104.5224035930334026, -253.8871293345330571, -324.9516776915779133 ) ) ;
#70544=CARTESIAN_POINT ( 'NONE',  ( -24.21168110473835355, -275.1569922701014548, -194.6736417776367318 ) ) ;
#70545=CARTESIAN_POINT ( 'NONE',  ( -111.7713335972482156, -274.2845451784580746, -253.5403743149537945 ) ) ;
#70546=CARTESIAN_POINT ( 'NONE',  ( -69.85430415644619018, -285.9805209788416391, -337.9475929042657754 ) ) ;
#70548=CARTESIAN_POINT ( 'NONE',  ( 82.65974748999957455, -298.7023692776643315, -193.0048141087816873 ) ) ;
#70549=CARTESIAN_POINT ( 'NONE',  ( 28.51143791346287060, -289.0663006257602774, -302.5727662283608197 ) ) ;
#70550=CARTESIAN_POINT ( 'NONE',  ( 38.56404369920143438, -289.2551970462341728, -265.8558366280998939 ) ) ;
#70551=CARTESIAN_POINT ( 'NONE',  ( 29.51492657283014154, -287.2995634214986467, -300.0515900678584558 ) ) ;
#70552=CARTESIAN_POINT ( 'NONE',  ( -113.4256106562333173, -284.2073298583755445, -258.5747209378415050 ) ) ;
#70553=CARTESIAN_POINT ( 'NONE',  ( -54.66097731631204226, -278.2258574878790114, -198.5693601604544085 ) ) ;
#70554=CARTESIAN_POINT ( 'NONE',  ( -88.56362733314142588, -287.1848107600865205, -216.6286357019850470 ) ) ;
#70555=CARTESIAN_POINT ( 'NONE',  ( 21.89775871414668984, -279.4230068406447458, -226.5061608593920255 ) ) ;
#70556=CARTESIAN_POINT ( 'NONE',  ( -110.6517425572639581, -279.9352688195127143, -265.1764139382601684 ) ) ;
#70557=CARTESIAN_POINT ( 'NONE',  ( -74.03876740984465243, -278.0463375420149532, -333.5379625905061971 ) ) ;
#70558=CARTESIAN_POINT ( 'NONE',  ( 0.5096636765602601260, -287.3546639809325711, -337.0189745407465693 ) ) ;
#70559=CARTESIAN_POINT ( 'NONE',  ( 4.466430853208652962, -283.3067222230526454, -334.8929082276620761 ) ) ;
#70560=CARTESIAN_POINT ( 'NONE',  ( -102.4697208731003002, -285.5813023078417814, -229.3993331460938521 ) ) ;
#70561=CARTESIAN_POINT ( 'NONE',  ( 22.58598527377359844, -282.2998419389450646, -312.0465174275540221 ) ) ;
#70565=CARTESIAN_POINT ( 'NONE',  ( -14.00086639007882283, -291.0334651374545842, -197.4460178483741402 ) ) ;
#70566=CARTESIAN_POINT ( 'NONE',  ( 9.645194837510528529, -273.7757085634275995, -214.1196150562338403 ) ) ;
#70567=CARTESIAN_POINT ( 'NONE',  ( -5.847044738855327495, -293.9974277255686275, -340.5138048082750970 ) ) ;
#70568=CARTESIAN_POINT ( 'NONE',  ( -53.57996250580212916, -287.7441635392947319, -342.2431504067977812 ) ) ;
#70569=CARTESIAN_POINT ( 'NONE',  ( -3.148454756994365500, -290.7501947822848933, -204.7196982342544800 ) ) ;
#70570=CARTESIAN_POINT ( 'NONE',  ( -68.91495787515356142, -290.6819340885292604, -336.6201543584406295 ) ) ;
#70572=CARTESIAN_POINT ( 'NONE',  ( -111.2068297495384712, -292.7192025140495275, -257.3632998353992889 ) ) ;
#70573=CARTESIAN_POINT ( 'NONE',  ( -61.08474469181454225, -289.7446191069391830, -198.9880305177079549 ) ) ;
#70574=CARTESIAN_POINT ( 'NONE',  ( 20.74891257241985087, -294.8983806487808579, -222.9019554595395505 ) ) ;
#70575=CARTESIAN_POINT ( 'NONE',  ( -22.42358052685474235, -287.1889949089036236, -198.6092940153311019 ) ) ;
#70576=CARTESIAN_POINT ( 'NONE',  ( -37.65514352323639713, -297.0561888998693689, -345.5399029053422737 ) ) ;
#70578=CARTESIAN_POINT ( 'NONE',  ( -3.323129829970142168, -276.4789223926416071, -203.1072809199720837 ) ) ;
#70579=CARTESIAN_POINT ( 'NONE',  ( -114.2394590020185916, -271.9367054066718197, -267.4891729012607016 ) ) ;
#70580=CARTESIAN_POINT ( 'NONE',  ( -11.11039515779607001, -272.6384964782828320, -201.0972641572010104 ) ) ;
#70581=CARTESIAN_POINT ( 'NONE',  ( -100.4078346138884825, -276.0953483828931780, -310.0045983443858404 ) ) ;
#70582=CARTESIAN_POINT ( 'NONE',  ( -110.2820711298114276, -273.8644937171459901, -262.1859860191879648 ) ) ;
#70583=CARTESIAN_POINT ( 'NONE',  ( 36.71864045377575536, -273.8897485159754979, -251.5549422005593954 ) ) ;
#70584=CARTESIAN_POINT ( 'NONE',  ( -80.48567844983057284, -297.0752971806296046, -329.9763178078274564 ) ) ;
#70585=DIRECTION ( 'NONE',  ( 0.000000000000000000, 0.000000000000000000, -1.000000000000000000 ) ) ;
#70586=CARTESIAN_POINT ( 'NONE',  ( -75.30315452064391479, -298.3352225353988842, -207.7601539663718881 ) ) ;
#70587=CARTESIAN_POINT ( 'NONE',  ( 104.1964229570258311, -299.5541904835127980, -197.2570935515975918 ) ) ;
#70588=CARTESIAN_POINT ( 'NONE',  ( 37.16323037804039586, -285.4269053045680380, -258.9868763035073016 ) ) ;
#70589=CARTESIAN_POINT ( 'NONE',  ( -70.46754843473301833, -297.6027994932200613, -205.2958560991954187 ) ) ;
#70590=CARTESIAN_POINT ( 'NONE',  ( 22.99188654876190441, -286.9117271993318354, -222.4980882501235442 ) ) ;
#70591=CARTESIAN_POINT ( 'NONE',  ( -23.31995607027534589, -288.5444258586746855, -346.1062668668715219 ) ) ;
#70592=CARTESIAN_POINT ( 'NONE',  ( -107.8886063954649757, -298.1879848769862633, -296.9948174597930688 ) ) ;
#70593=CARTESIAN_POINT ( 'NONE',  ( 20.22756712470414087, -292.2135310225754097, -318.1712413682008673 ) ) ;
#70594=CARTESIAN_POINT ( 'NONE',  ( 24.11978028618081638, -281.3644002837964422, -316.4766820177440536 ) ) ;
#70595=CARTESIAN_POINT ( 'NONE',  ( -20.19161114001082069, -283.7666405000204009, -195.3683826091709363 ) ) ;
#70597=CARTESIAN_POINT ( 'NONE',  ( -53.51085341094929504, -288.0591590709166212, -341.9550352222351535 ) ) ;
#70599=CARTESIAN_POINT ( 'NONE',  ( -34.52779919839132816, -287.0167631635330849, -345.3592581997543220 ) ) ;
#70600=CARTESIAN_POINT ( 'NONE',  ( -35.13795689164769698, -299.6803177653247872, -196.5604998867146662 ) ) ;
#70601=CARTESIAN_POINT ( 'NONE',  ( -31.13982462235754767, -281.5541829127319033, -194.1501602831974367 ) ) ;
#70602=CARTESIAN_POINT ( 'NONE',  ( -76.25493553000536906, -293.5892621223344463, -334.9521914411866419 ) ) ;
#70603=CARTESIAN_POINT ( 'NONE',  ( -13.52936602132302646, -282.7343400366372066, -339.4217709840478960 ) ) ;
#70604=CARTESIAN_POINT ( 'NONE',  ( -113.9430046164710291, -296.6209616882620139, -278.1867269155716826 ) ) ;
#70605=CARTESIAN_POINT ( 'NONE',  ( -39.20508215459190637, -299.5485054782038787, -196.6788177819891814 ) ) ;
#70606=CARTESIAN_POINT ( 'NONE',  ( 37.41608068887489935, -283.4749831315580195, -264.3382570356354790 ) ) ;
#70608=CARTESIAN_POINT ( 'NONE',  ( -44.58045220042586010, -297.0171962089432895, -197.4339045375737953 ) ) ;
#70611=CARTESIAN_POINT ( 'NONE',  ( -76.97965838967209606, -285.5654508912245433, -333.6731560313812111 ) ) ;
#70613=CARTESIAN_POINT ( 'NONE',  ( 25.18497378105905682, -279.6952119285918457, -320.2651865833026363 ) ) ;
#70614=CARTESIAN_POINT ( 'NONE',  ( 0.9576560570261686278, -275.7521778843654943, -337.0346634714132961 ) ) ;
#70615=CARTESIAN_POINT ( 'NONE',  ( -20.07010538936605926, -292.1135301807131555, -199.3814768179931320 ) ) ;
#70616=CARTESIAN_POINT ( 'NONE',  ( -48.41393097179969374, -284.7157729575237113, -343.2179190051014075 ) ) ;
#70617=CARTESIAN_POINT ( 'NONE',  ( 19.81396966363418954, -277.8063247213278828, -317.0679731432012431 ) ) ;
#70618=CARTESIAN_POINT ( 'NONE',  ( -67.63096305686403298, -284.8671335737280401, -340.5121468077363716 ) ) ;
#70619=CARTESIAN_POINT ( 'NONE',  ( -61.68079291410877119, -282.1703689347894510, -339.6587028862649049 ) ) ;
#70620=CARTESIAN_POINT ( 'NONE',  ( -43.95207306985640372, -281.9688793268086329, -195.6013848918130975 ) ) ;
#70621=CARTESIAN_POINT ( 'NONE',  ( 37.28470295454496153, -275.4814433800626148, -251.3900882931308729 ) ) ;
#70622=CARTESIAN_POINT ( 'NONE',  ( 37.90522360908004629, -275.5905612598006087, -286.7598025223084051 ) ) ;
#70623=CARTESIAN_POINT ( 'NONE',  ( -109.6929327665311718, -298.2450868897143437, -287.9251779765749006 ) ) ;
#70627=CARTESIAN_POINT ( 'NONE',  ( -94.66276608479341803, -294.0115916068578485, -319.9050467741159878 ) ) ;
#70628=CARTESIAN_POINT ( 'NONE',  ( 35.70455869101828483, -275.0401079366844783, -268.8669580202108591 ) ) ;
#70629=CARTESIAN_POINT ( 'NONE',  ( 34.83696766509952170, -295.3889646272189111, -295.2809408000693452 ) ) ;
#70630=CARTESIAN_POINT ( 'NONE',  ( -0.8815773038446524934, -295.7841761692653222, -337.7455661287014550 ) ) ;
#70631=CARTESIAN_POINT ( 'NONE',  ( -71.06925274681060500, -293.6060966429259338, -203.5593169245541390 ) ) ;
#70632=CARTESIAN_POINT ( 'NONE',  ( -96.74345866326923726, -275.9274016480878799, -315.8744073948667506 ) ) ;
#70633=CARTESIAN_POINT ( 'NONE',  ( -110.9115808234451919, -280.3255004165364426, -281.7095475203002479 ) ) ;
#70634=CARTESIAN_POINT ( 'NONE',  ( -111.4822010659440963, -294.7254598494309903, -263.1360414614928231 ) ) ;
#70635=CARTESIAN_POINT ( 'NONE',  ( -13.78315774987723508, -284.6100173665847706, -342.3701490817223316 ) ) ;
#70636=CARTESIAN_POINT ( 'NONE',  ( -85.92074389041499671, -284.2809209862342072, -215.3906168898256510 ) ) ;
#70637=CARTESIAN_POINT ( 'NONE',  ( 175.7436469805359138, 241.6859982463862764, -179.0910351515699404 ) ) ;
#70639=CARTESIAN_POINT ( 'NONE',  ( -108.3850958888772453, -284.4421330787102988, -253.4276063474368925 ) ) ;
#70641=CARTESIAN_POINT ( 'NONE',  ( 22.29162071927039079, -283.2812166626516159, -318.6038246925293720 ) ) ;
#70642=CARTESIAN_POINT ( 'NONE',  ( -85.25255792420603029, -284.2018111161890488, -210.5902352494255183 ) ) ;
#70643=CARTESIAN_POINT ( 'NONE',  ( -113.0065967426592692, -279.6558260396728883, -257.4133910178989595 ) ) ;
#70644=CARTESIAN_POINT ( 'NONE',  ( -67.41735561851342595, -278.9596546773233854, -340.4907315612996968 ) ) ;
#70645=CARTESIAN_POINT ( 'NONE',  ( -19.78756432573599255, -280.9233879431179162, -195.4387709399019286 ) ) ;
#70646=CARTESIAN_POINT ( 'NONE',  ( -67.68488546085839630, -271.1237833571632905, -207.2794874003663779 ) ) ;
#70647=CARTESIAN_POINT ( 'NONE',  ( 154.9793621001980171, 206.4414210594577810, -217.3080705048732000 ) ) ;
#70648=CARTESIAN_POINT ( 'NONE',  ( -65.27622544172163543, -275.6864015259907319, -200.9233048794513081 ) ) ;
#70649=CARTESIAN_POINT ( 'NONE',  ( -56.72725910259299553, -169.1093196520039896, -364.2234470880441677 ) ) ;
#70650=CARTESIAN_POINT ( 'NONE',  ( -16.43746510500518454, -278.3437527998024734, -198.7031822165723440 ) ) ;
#70651=CARTESIAN_POINT ( 'NONE',  ( -33.61182275531538721, -293.8586316445739044, -194.4660454823589646 ) ) ;
#70652=CARTESIAN_POINT ( 'NONE',  ( -73.35984233925489661, -294.8920769460565907, -333.9739005027352050 ) ) ;
#70653=CARTESIAN_POINT ( 'NONE',  ( -91.55961797117340950, -289.3066363431200898, -325.0249355406274390 ) ) ;
#70655=CARTESIAN_POINT ( 'NONE',  ( -108.3343685712820843, -295.4897563664371205, -241.9586675408789631 ) ) ;
#70656=CARTESIAN_POINT ( 'NONE',  ( -44.07732395128466862, -284.3654367520975370, -196.8691334757363336 ) ) ;
#70657=CARTESIAN_POINT ( 'NONE',  ( -104.6866562303662960, -292.8271419034650762, -239.1277645757311348 ) ) ;
#70658=CARTESIAN_POINT ( 'NONE',  ( -91.89848163743893394, -286.5684738427502793, -221.0440507880120720 ) ) ;
#70660=CARTESIAN_POINT ( 'NONE',  ( -97.28736398845788358, -292.1376555841567892, -222.4097092588899898 ) ) ;
#70661=CARTESIAN_POINT ( 'NONE',  ( 33.02040192359089588, -282.3043472551283912, -290.0375769284212311 ) ) ;
#70662=CARTESIAN_POINT ( 'NONE',  ( -5.974399706019373646, -293.4438547410977662, -340.2474627434253307 ) ) ;
#70663=CARTESIAN_POINT ( 'NONE',  ( -34.66219235671446341, -289.8221113137282714, -347.1529082926700767 ) ) ;
#70664=CARTESIAN_POINT ( 'NONE',  ( -113.6060034133675032, -291.1765843419334487, -259.8080197763021602 ) ) ;
#70665=CARTESIAN_POINT ( 'NONE',  ( 34.96066830824933191, -287.8528494374757543, -280.5202924721663749 ) ) ;
#70668=CARTESIAN_POINT ( 'NONE',  ( -111.0777919943166836, -298.6339279672222915, -252.9457729987560413 ) ) ;
#70669=CARTESIAN_POINT ( 'NONE',  ( -30.52231065812785005, -296.8206805055173731, -193.8557524509169241 ) ) ;
#70670=CARTESIAN_POINT ( 'NONE',  ( 32.96382175207060072, -280.3404865373345842, -249.8539962539578028 ) ) ;
#70672=CARTESIAN_POINT ( 'NONE',  ( 7.922900236742358437, -297.9535122079532243, -193.4678911002017969 ) ) ;
#70673=CARTESIAN_POINT ( 'NONE',  ( -89.00156356406070302, -294.2738993897837645, -322.9872633757727272 ) ) ;
#70674=CARTESIAN_POINT ( 'NONE',  ( 17.29411997095717268, -278.0188502902738605, -320.3089888615491532 ) ) ;
#70675=CARTESIAN_POINT ( 'NONE',  ( -59.82760629727908253, -271.8974409596727355, -199.5595195205677896 ) ) ;
#70676=CARTESIAN_POINT ( 'NONE',  ( -7.814561675065936797, -295.8614746109129214, -337.5705935758317651 ) ) ;
#70677=CARTESIAN_POINT ( 'NONE',  ( -4.184601490418486947, -295.6840477155105305, -335.7573827203992209 ) ) ;
#70678=CARTESIAN_POINT ( 'NONE',  ( -22.23600029014999180, -296.4619124217902595, -345.0488562389193703 ) ) ;
#70679=CARTESIAN_POINT ( 'NONE',  ( -110.8334523444457744, -270.7850977723512642, -253.7067142414082355 ) ) ;
#70680=CARTESIAN_POINT ( 'NONE',  ( -0.04606956585158543394, -293.2141482659956750, -207.4887980860360983 ) ) ;
#70681=CARTESIAN_POINT ( 'NONE',  ( -85.71451769584137992, -274.2046527044727213, -210.6599509876731133 ) ) ;
#70682=CARTESIAN_POINT ( 'NONE',  ( -109.8542297915555821, -289.2948059940875396, -257.5283358732006604 ) ) ;
#70683=CARTESIAN_POINT ( 'NONE',  ( 50.62885399555703003, -301.1535713209074743, -195.3311200258940801 ) ) ;
#70684=CARTESIAN_POINT ( 'NONE',  ( -58.11103645772325166, -274.2832579749527895, -196.2236088678313308 ) ) ;
#70685=CARTESIAN_POINT ( 'NONE',  ( -94.47051604516552459, -297.5274950952226050, -224.8816074443593891 ) ) ;
#70686=CARTESIAN_POINT ( 'NONE',  ( 18.88425334251419940, -282.8367697728737653, -220.1715236988281674 ) ) ;
#70687=CARTESIAN_POINT ( 'NONE',  ( 36.71023826732177753, -280.4791589901851125, -289.5863278382886392 ) ) ;
#70688=CARTESIAN_POINT ( 'NONE',  ( -103.5223005592907413, -277.3887585378208200, -309.6247324694608096 ) ) ;
#70689=CARTESIAN_POINT ( 'NONE',  ( 38.00683522936126479, -279.8041368919586489, -258.6587801150954533 ) ) ;
#70690=CARTESIAN_POINT ( 'NONE',  ( 23.13230107297217231, -278.9442864628056213, -225.7189450079954440 ) ) ;
#70692=CARTESIAN_POINT ( 'NONE',  ( -83.54657151150803429, -271.9786011799494645, -213.0856016090108938 ) ) ;
#70693=CARTESIAN_POINT ( 'NONE',  ( -109.5194072967893817, -280.8166845782808991, -249.7960249768669314 ) ) ;
#70696=CARTESIAN_POINT ( 'NONE',  ( 52.12392687579448136, -297.3974167468510927, -194.4008023326589125 ) ) ;
#70697=CARTESIAN_POINT ( 'NONE',  ( 35.12940740477638712, -291.3072444358027155, -249.6659116943681056 ) ) ;
#70698=CARTESIAN_POINT ( 'NONE',  ( -0.8038585024801646606, -292.5237588303530174, -202.5821674939128343 ) ) ;
#70699=CARTESIAN_POINT ( 'NONE',  ( 37.10481316069009949, -277.4193302802048606, -259.9810849550235616 ) ) ;
#70700=CARTESIAN_POINT ( 'NONE',  ( -10.75812699870826528, -272.3985159328415762, -200.1748887448128755 ) ) ;
#70701=CARTESIAN_POINT ( 'NONE',  ( 133.0872704186301405, -299.5541904835127980, -195.3611179825600175 ) ) ;
#70702=CARTESIAN_POINT ( 'NONE',  ( 28.51897698165462813, -283.9631852285235709, -307.5040850942365864 ) ) ;
#70704=CARTESIAN_POINT ( 'NONE',  ( -10.29800412807189858, -284.4048991122417647, -200.3929035370040594 ) ) ;
#70705=CARTESIAN_POINT ( 'NONE',  ( 145.2857639756989272, -299.5541904835127980, -197.7582414438974183 ) ) ;
#70706=CARTESIAN_POINT ( 'NONE',  ( -38.36312993873905697, -293.8601601522237843, -343.7510845122176875 ) ) ;
#70707=CARTESIAN_POINT ( 'NONE',  ( -7.741012508047727003, -284.5838641656993104, -202.2827456846001724 ) ) ;
#70709=CARTESIAN_POINT ( 'NONE',  ( 15.71356215118052013, -292.3014939926353577, -323.4448647308847171 ) ) ;
#70710=CARTESIAN_POINT ( 'NONE',  ( -87.87699077656239410, -282.2230783892252362, -327.6059123063656102 ) ) ;
#70711=CARTESIAN_POINT ( 'NONE',  ( -35.66482983202826773, -281.6736341949624602, -196.5676293687050133 ) ) ;
#70712=CARTESIAN_POINT ( 'NONE',  ( 38.69836476072104858, -288.8791217104626980, -280.0576190536216927 ) ) ;
#70713=CARTESIAN_POINT ( 'NONE',  ( 15.03858046935243031, -280.5651228866703377, -325.4090990231875935 ) ) ;
#70714=CARTESIAN_POINT ( 'NONE',  ( 19.51519123708373726, -286.9046031848852181, -224.5560103911538761 ) ) ;
#70715=CARTESIAN_POINT ( 'NONE',  ( -98.49328912324190810, -280.5425154618237684, -229.3333581189755535 ) ) ;
#70716=CARTESIAN_POINT ( 'NONE',  ( -93.72395175566229852, -278.6952905057843850, -317.0030921002418154 ) ) ;
#70717=CARTESIAN_POINT ( 'NONE',  ( -1.768764252945906001, -288.5010164096829612, -203.9309061948313229 ) ) ;
#70719=CARTESIAN_POINT ( 'NONE',  ( -34.75730480598763705, -297.9169931902062558, -193.3611886416082939 ) ) ;
#70720=CARTESIAN_POINT ( 'NONE',  ( -94.71999691202900351, -293.1946494561245800, -222.5962301135205337 ) ) ;
#70722=CARTESIAN_POINT ( 'NONE',  ( -95.99890600148557951, -275.6948066931273615, -223.6242672951989618 ) ) ;
#70724=CARTESIAN_POINT ( 'NONE',  ( 33.01491732840578663, -273.2091214656009583, -243.9040810211828330 ) ) ;
#70725=CARTESIAN_POINT ( 'NONE',  ( -65.32883455222767566, -293.8117891581078993, -341.2494538634662717 ) ) ;
#70726=CARTESIAN_POINT ( 'NONE',  ( -34.47060486770152465, -297.5967001460852543, -197.2998270489071899 ) ) ;
#70727=CARTESIAN_POINT ( 'NONE',  ( 18.36221253671129361, -289.7540299844526430, -318.6846380148112416 ) ) ;
#70728=CARTESIAN_POINT ( 'NONE',  ( 11.96443253659156269, -282.5089370640034190, -215.1625736811821241 ) ) ;
#70729=CARTESIAN_POINT ( 'NONE',  ( -84.78451456822662635, -291.1165543216309288, -330.3267409472321106 ) ) ;
#70730=CARTESIAN_POINT ( 'NONE',  ( -111.5205782233828273, -292.1037796233807740, -251.5788515009789137 ) ) ;
#70731=CARTESIAN_POINT ( 'NONE',  ( -24.83265226918851809, -288.2117554175019336, -196.3589449734167829 ) ) ;
#70732=CARTESIAN_POINT ( 'NONE',  ( 19.15871865419534359, -281.0062233138215788, -218.0476141624534989 ) ) ;
#70733=CARTESIAN_POINT ( 'NONE',  ( 26.86906999661741580, -292.1639613655659105, -310.2876393133010424 ) ) ;
#70734=CARTESIAN_POINT ( 'NONE',  ( 8.548240937587799237, -280.4943831958558462, -208.4635080494362853 ) ) ;
#70735=CARTESIAN_POINT ( 'NONE',  ( -11.07496819274521904, -276.2584696785129950, -200.8732889035858022 ) ) ;
#70736=CARTESIAN_POINT ( 'NONE',  ( -92.08974858914540107, -275.6948066931273047, -226.7417163044926838 ) ) ;
#70737=CARTESIAN_POINT ( 'NONE',  ( 27.64765862432134469, -273.2700632916935319, -230.8859052190877605 ) ) ;
#70739=CARTESIAN_POINT ( 'NONE',  ( 31.41037744323099545, -281.3905397257452137, -295.2319184282449669 ) ) ;
#70740=CARTESIAN_POINT ( 'NONE',  ( -70.11712441390601214, -278.6794192926264486, -339.6126107171586455 ) ) ;
#70741=CARTESIAN_POINT ( 'NONE',  ( -90.56522099978477058, -274.5934213320003892, -219.6623275673659634 ) ) ;
#70742=CARTESIAN_POINT ( 'NONE',  ( -23.81554843122183840, -285.2795309959327597, -194.7434271090556024 ) ) ;
#70743=CARTESIAN_POINT ( 'NONE',  ( -108.3740525596705595, -292.5841545060434328, -249.5223453703365237 ) ) ;
#70744=CARTESIAN_POINT ( 'NONE',  ( -18.76493754809575165, -275.8874733854373176, -196.4057545819365771 ) ) ;
#70745=CARTESIAN_POINT ( 'NONE',  ( -91.82967052955407894, -274.6097341848593487, -216.6548859997681404 ) ) ;
#70747=CARTESIAN_POINT ( 'NONE',  ( 11.74613352572937686, -276.1813034930604545, -324.4610386118191059 ) ) ;
#70748=CARTESIAN_POINT ( 'NONE',  ( -107.7024545047438124, -298.2193793716484720, -295.9965257390982174 ) ) ;
#70749=CARTESIAN_POINT ( 'NONE',  ( -97.21790990838889002, -283.1666775140588470, -225.4738376924498766 ) ) ;
#70750=CARTESIAN_POINT ( 'NONE',  ( -11.15645225876424185, -292.0508542489702677, -197.9167176020374086 ) ) ;
#70751=CARTESIAN_POINT ( 'NONE',  ( 21.15997851667113139, -272.9321101434353523, -223.9790298987078643 ) ) ;
#70752=CARTESIAN_POINT ( 'NONE',  ( 7.480570308289862247, -290.0526243487146871, -332.0492819720870443 ) ) ;
#70754=CARTESIAN_POINT ( 'NONE',  ( -110.2790591626303609, -289.5693331432657374, -262.9876703303661429 ) ) ;
#70756=CARTESIAN_POINT ( 'NONE',  ( -111.0595049218839279, -289.3812287864160453, -250.2045108625517855 ) ) ;
#70757=CARTESIAN_POINT ( 'NONE',  ( -100.3243372570148324, -289.7104707549527234, -307.4103441977669036 ) ) ;
#70759=CARTESIAN_POINT ( 'NONE',  ( 11.86865752226332660, -287.7967430556263935, -211.4714849669444163 ) ) ;
#70760=CARTESIAN_POINT ( 'NONE',  ( -107.1355745642640898, -278.5991251391711785, -291.9990437630934252 ) ) ;
#70762=CARTESIAN_POINT ( 'NONE',  ( -50.42835683319628970, -294.1356815582636841, -345.9809241825311688 ) ) ;
#70763=CARTESIAN_POINT ( 'NONE',  ( -74.21979752927676088, -284.1801574528889773, -337.8988115726390902 ) ) ;
#70764=CARTESIAN_POINT ( 'NONE',  ( -106.6619132904246214, -285.3150219072456366, -236.8879595035300554 ) ) ;
#70765=CARTESIAN_POINT ( 'NONE',  ( -6.020023963921404153, -282.9621175227376284, -336.3372867996187097 ) ) ;
#70766=CARTESIAN_POINT ( 'NONE',  ( 121.7669983244749403, 149.6016541078746798, -263.6324895168810372 ) ) ;
#70767=CARTESIAN_POINT ( 'NONE',  ( -110.7434605763195350, -265.2408335553506049, -306.4457901866108500 ) ) ;
#70768=CARTESIAN_POINT ( 'NONE',  ( -13.40524764562645998, -91.92062792358137813, -356.3535239457285684 ) ) ;
#70769=CARTESIAN_POINT ( 'NONE',  ( 21.61736411087281695, -274.1437539661689584, -227.0433332815328527 ) ) ;
#70770=CARTESIAN_POINT ( 'NONE',  ( -29.94506394337190969, -273.0682956552009273, -197.4261068655856093 ) ) ;
#70771=CARTESIAN_POINT ( 'NONE',  ( -97.36337231765800482, -295.4141523037879438, -318.5164254622376916 ) ) ;
#70772=CARTESIAN_POINT ( 'NONE',  ( -81.75305709561430945, -219.5167969555488696, -349.4486404927797594 ) ) ;
#70773=CARTESIAN_POINT ( 'NONE',  ( 28.66199125000223802, -274.7438343475895408, -309.0497596781670495 ) ) ;
#70774=CARTESIAN_POINT ( 'NONE',  ( -84.88375982183343638, -299.2492189638595619, -213.2797923915757963 ) ) ;
#70775=CARTESIAN_POINT ( 'NONE',  ( -103.8424724307707834, -292.0465230206620504, -239.5086730910153960 ) ) ;
#70777=CARTESIAN_POINT ( 'NONE',  ( -107.5626621740012610, -297.8917778681564528, -239.2161547970895015 ) ) ;
#70778=CARTESIAN_POINT ( 'NONE',  ( 30.54468721774808770, -288.4071901495208863, -297.5055009630654013 ) ) ;
#70779=CARTESIAN_POINT ( 'NONE',  ( -114.1765953379295553, -297.3643426482988161, -269.6143261189695863 ) ) ;
#70780=CARTESIAN_POINT ( 'NONE',  ( -61.56623761386740057, -295.8508433272298248, -343.4421396056974913 ) ) ;
#70781=CARTESIAN_POINT ( 'NONE',  ( 34.48279183177873364, -293.5457952988538750, -257.2439245673625692 ) ) ;
#70783=CARTESIAN_POINT ( 'NONE',  ( 36.50367686172460679, -277.6770576018200813, -286.4271100973249418 ) ) ;
#70784=CARTESIAN_POINT ( 'NONE',  ( 37.92577506058935199, -280.8594089999433550, -254.3502113396222626 ) ) ;
#70785=CARTESIAN_POINT ( 'NONE',  ( 22.46608172164806660, -275.9050657113726288, -228.0731430680824872 ) ) ;
#70786=CARTESIAN_POINT ( 'NONE',  ( -18.81897362504284743, -276.0474604769079860, -196.6122938103376896 ) ) ;
#70787=CARTESIAN_POINT ( 'NONE',  ( -96.65031552451543462, -275.9373209348626688, -316.8465452376109397 ) ) ;
#70788=CARTESIAN_POINT ( 'NONE',  ( -35.15223256983011879, -298.7316880494328188, -197.2589340308238377 ) ) ;
#70789=CARTESIAN_POINT ( 'NONE',  ( -108.0202760814093637, -295.3957475003086302, -249.8693191578521464 ) ) ;
#70791=CARTESIAN_POINT ( 'NONE',  ( -97.65256745355323176, -279.6842546397919023, -222.5895135921271617 ) ) ;
#70792=CARTESIAN_POINT ( 'NONE',  ( -64.33116664940294527, -277.5809682468732262, -338.2422917424806883 ) ) ;
#70793=CARTESIAN_POINT ( 'NONE',  ( 9.521973557649090480, -285.3664268247834457, -209.8872032745990737 ) ) ;
#70794=CARTESIAN_POINT ( 'NONE',  ( -72.44761772685525614, -299.5891825052127615, -203.8386099904832065 ) ) ;
#70796=CARTESIAN_POINT ( 'NONE',  ( 32.46461100160329494, -287.0409532486501121, -292.4312667663220395 ) ) ;
#70797=CARTESIAN_POINT ( 'NONE',  ( -92.95524589532598725, -277.4797638914051845, -221.5042826305259496 ) ) ;
#70798=CARTESIAN_POINT ( 'NONE',  ( -108.8580466930563233, -277.3538706080149154, -253.0179033753887552 ) ) ;
#70799=CARTESIAN_POINT ( 'NONE',  ( -36.19540709172365922, -281.1175158213353598, -344.7922956809714492 ) ) ;
#70800=CARTESIAN_POINT ( 'NONE',  ( -9.061834272863206863, -288.4220971198014922, -200.8834562642012145 ) ) ;
#70801=CARTESIAN_POINT ( 'NONE',  ( 12.02606585383540150, -277.5528384434420559, -324.7435777997233117 ) ) ;
#70803=CARTESIAN_POINT ( 'NONE',  ( -96.77930032168920604, -293.1791205013205399, -224.6000568379405706 ) ) ;
#70804=CARTESIAN_POINT ( 'NONE',  ( -48.36937523186626464, -275.4303816882110141, -345.5965130343774376 ) ) ;
#70806=CARTESIAN_POINT ( 'NONE',  ( 35.20830795973833460, -276.3270031044157236, -279.7311829732614115 ) ) ;
#70807=CARTESIAN_POINT ( 'NONE',  ( 33.58899650509938084, -283.2290831287344872, -245.3288222576561850 ) ) ;
#70811=CARTESIAN_POINT ( 'NONE',  ( 36.70217038495741946, -289.6642440373236695, -285.4216438930553181 ) ) ;
#70812=CARTESIAN_POINT ( 'NONE',  ( -15.02810889987506648, -292.7631167202657707, -342.0183686775097840 ) ) ;
#70814=CARTESIAN_POINT ( 'NONE',  ( -13.89234434362371395, -273.0477289436876731, -200.7093327168589951 ) ) ;
#70815=CARTESIAN_POINT ( 'NONE',  ( 34.50961580373898840, -291.4494648481593231, -251.6995563758633807 ) ) ;
#70816=CARTESIAN_POINT ( 'NONE',  ( 201.7194887906492795, 294.2213704821156739, -83.28174295417332473 ) ) ;
#70817=CARTESIAN_POINT ( 'NONE',  ( -16.79453476385504018, -290.7927503646538980, -196.8728757492164902 ) ) ;
#70818=CARTESIAN_POINT ( 'NONE',  ( -81.08410058457873504, -285.2573002304844181, -329.8640910098963559 ) ) ;
#70819=CARTESIAN_POINT ( 'NONE',  ( 4.638762607568192031, -284.8498623947787110, -206.9611264115397091 ) ) ;
#70820=CARTESIAN_POINT ( 'NONE',  ( -81.84925480297376055, -286.8573669588631105, -211.7569159802048375 ) ) ;
#70821=CARTESIAN_POINT ( 'NONE',  ( -97.49451986551379434, -285.9341491107848583, -228.6947617901457761 ) ) ;
#70822=CARTESIAN_POINT ( 'NONE',  ( -100.3234184067648300, -293.0888348299243376, -228.8946195672068598 ) ) ;
#70823=CARTESIAN_POINT ( 'NONE',  ( 35.89564589079301982, -273.3949467998783120, -251.7706540483175672 ) ) ;
#70824=CARTESIAN_POINT ( 'NONE',  ( 26.91057509555442451, -275.3277704181090257, -227.9654882538820857 ) ) ;
#70825=CARTESIAN_POINT ( 'NONE',  ( -99.50999185160974037, -288.0540628125497165, -313.3078024046383803 ) ) ;
#70826=CARTESIAN_POINT ( 'NONE',  ( 12.70461835195821187, -276.3762486724124869, -328.8792007142631064 ) ) ;
#70827=CARTESIAN_POINT ( 'NONE',  ( -81.09904172917407550, -297.6298277862287023, -330.8354253859787377 ) ) ;
#70829=DIRECTION ( 'NONE',  ( 1.000000000000000000, 0.000000000000000000, 0.000000000000000000 ) ) ;
#70830=CARTESIAN_POINT ( 'NONE',  ( -109.9884243026998689, -283.0869569537228472, -281.8100087106455476 ) ) ;
#70831=CARTESIAN_POINT ( 'NONE',  ( -69.09190519811453157, -277.6344828303724626, -202.3991451189241957 ) ) ;
#70832=CARTESIAN_POINT ( 'NONE',  ( 133.0872704186301405, -299.5541904835127980, -195.3611179825600175 ) ) ;
#70833=CARTESIAN_POINT ( 'NONE',  ( 37.54211186496195296, -273.8469372919240072, -255.6940645699230572 ) ) ;
#70834=CARTESIAN_POINT ( 'NONE',  ( -18.99936815586674754, -276.1583093663208501, -341.1244667279741520 ) ) ;
#70835=CARTESIAN_POINT ( 'NONE',  ( -34.25294064596364763, -296.5327388078561626, -343.9896947619949401 ) ) ;
#70836=CARTESIAN_POINT ( 'NONE',  ( 24.35129957681044033, -279.8646267406712127, -224.8038320897036613 ) ) ;
#70837=CARTESIAN_POINT ( 'NONE',  ( 12.52383084865697604, -295.2782116472359917, -324.0667909051300057 ) ) ;
#70838=CARTESIAN_POINT ( 'NONE',  ( 3.975161723384856849, -295.8236933992315016, -334.8146109976244134 ) ) ;
#70839=CARTESIAN_POINT ( 'NONE',  ( -110.3626861462309137, -272.2548568503066235, -267.6322362053812185 ) ) ;
#70840=CARTESIAN_POINT ( 'NONE',  ( -108.4760689522130832, -292.8595474916429566, -246.5934462369953337 ) ) ;
#70841=CARTESIAN_POINT ( 'NONE',  ( -7.345088173612762894, -286.6013459820299545, -199.3875874785503015 ) ) ;
#70842=CARTESIAN_POINT ( 'NONE',  ( -1.858659863862177630, -272.6567042821487235, -203.4189090541416931 ) ) ;
#70843=CARTESIAN_POINT ( 'NONE',  ( 9.812428825423710421, -286.5147359564604699, -209.4883972685940705 ) ) ;
#70844=CARTESIAN_POINT ( 'NONE',  ( -95.23176189144186310, -281.1843245766279438, -223.2380073489340191 ) ) ;
#70845=CARTESIAN_POINT ( 'NONE',  ( -37.26864129253610258, -285.1117984819755975, -197.1133809304161559 ) ) ;
#70847=CARTESIAN_POINT ( 'NONE',  ( -102.0851540078492832, -288.0449517654854503, -308.3226612088314482 ) ) ;
#70848=CARTESIAN_POINT ( 'NONE',  ( -109.0101294763935016, -268.7602059993127455, -295.2240039188629339 ) ) ;
#70849=CARTESIAN_POINT ( 'NONE',  ( -33.22892778159213378, -285.6128458873258751, -197.3655671618930967 ) ) ;
#70851=CARTESIAN_POINT ( 'NONE',  ( 4.427753012850422110, -283.4451193332757271, -334.8299503909703390 ) ) ;
#70852=CARTESIAN_POINT ( 'NONE',  ( -47.69974089432111697, -290.9824113499088867, -194.2448091947306921 ) ) ;
#70853=CARTESIAN_POINT ( 'NONE',  ( -111.9386192217766620, -280.3495570346349268, -254.7501178991218183 ) ) ;
#70854=CARTESIAN_POINT ( 'NONE',  ( -113.5861292134884764, -279.7799453703643735, -277.3031037038877571 ) ) ;
#70855=CARTESIAN_POINT ( 'NONE',  ( 33.64965152270030302, -281.6105199244289565, -287.4209966694936611 ) ) ;
#70856=CARTESIAN_POINT ( 'NONE',  ( -3.216824501555996640, -276.5029539138312202, -203.5597764831137795 ) ) ;
#70857=CARTESIAN_POINT ( 'NONE',  ( -92.69700478724686832, -295.8189102268943316, -323.8848533351208516 ) ) ;
#70858=CARTESIAN_POINT ( 'NONE',  ( -111.3270007188919664, -288.7049181055403437, -260.0780928245881682 ) ) ;
#70859=CARTESIAN_POINT ( 'NONE',  ( -90.64139173792274562, -294.7498978232420654, -320.7668231668674821 ) ) ;
#70862=CARTESIAN_POINT ( 'NONE',  ( 20.48585876962583185, -284.1228759773125034, -317.2564523177530305 ) ) ;
#70863=CARTESIAN_POINT ( 'NONE',  ( -69.73726499790593891, -295.1576538710190789, -335.8028085447425042 ) ) ;
#70864=CARTESIAN_POINT ( 'NONE',  ( 39.19467391036910442, -294.7026612976429192, -276.0026567837508651 ) ) ;
#70865=CARTESIAN_POINT ( 'NONE',  ( -16.09496319479997339, -283.4214472279232950, -340.3073032797045130 ) ) ;
#70866=CARTESIAN_POINT ( 'NONE',  ( -10.41887150142800245, -273.4536276322706954, -198.4158897540949340 ) ) ;
#70867=CARTESIAN_POINT ( 'NONE',  ( -112.7663882200000387, -291.0151208418662350, -285.4087876665742556 ) ) ;
#70868=CARTESIAN_POINT ( 'NONE',  ( -43.54118546448030003, -284.1143461959666752, -194.7979735607809175 ) ) ;
#70869=CARTESIAN_POINT ( 'NONE',  ( -110.4121741973763733, -291.1922175175238294, -245.9775461755935453 ) ) ;
#70870=CARTESIAN_POINT ( 'NONE',  ( 30.99288311759143966, -287.5403570270709679, -244.4798690943914607 ) ) ;
#70873=CARTESIAN_POINT ( 'NONE',  ( -111.0016612856833831, -271.0675853585269692, -270.3422158909584709 ) ) ;
#70874=CARTESIAN_POINT ( 'NONE',  ( 22.86789198823231928, -283.7044044627420476, -317.2598756660011077 ) ) ;
#70875=CARTESIAN_POINT ( 'NONE',  ( 21.31550574532286291, -284.4094976428775681, -223.6242672951989618 ) ) ;
#70877=CARTESIAN_POINT ( 'NONE',  ( 0.5715380142630172022, -279.4903416938436180, -207.5583266017104904 ) ) ;
#70878=CARTESIAN_POINT ( 'NONE',  ( -9.223495967937791917, -276.3611309706924999, -342.0208059970449881 ) ) ;
#70879=CARTESIAN_POINT ( 'NONE',  ( -57.05930384398344302, -279.3071096992368325, -342.6038788174282672 ) ) ;
#70880=CARTESIAN_POINT ( 'NONE',  ( -110.4560292262735146, -273.1165755189331890, -283.8932947766008397 ) ) ;
#70881=CARTESIAN_POINT ( 'NONE',  ( 39.03029897396627490, -280.1575556320187843, -272.7950539921042719 ) ) ;
#70882=CARTESIAN_POINT ( 'NONE',  ( -70.69524898940100854, -283.6302444693379812, -203.5682154360150946 ) ) ;
#70883=CARTESIAN_POINT ( 'NONE',  ( -110.9809931515036681, -298.0740481028470867, -289.1546767135573646 ) ) ;
#70884=CARTESIAN_POINT ( 'NONE',  ( 28.45269661009361073, -294.4754240874830771, -302.2439228450415385 ) ) ;
#70887=CARTESIAN_POINT ( 'NONE',  ( -108.2057804588883840, -288.9790778856013276, -290.0302338702121574 ) ) ;
#70888=CARTESIAN_POINT ( 'NONE',  ( -10.39112158241530715, -275.0460359887375148, -198.2837869965204618 ) ) ;
#70889=CARTESIAN_POINT ( 'NONE',  ( -108.5348967160139750, -272.7650774939410780, -254.2202146747527536 ) ) ;
#70893=CARTESIAN_POINT ( 'NONE',  ( 34.86921037486619213, -282.4657665448449961, -257.7195010579127938 ) ) ;
#70894=CARTESIAN_POINT ( 'NONE',  ( -86.17093577143498351, -281.1462028920039984, -212.0715622585161952 ) ) ;
#70895=CARTESIAN_POINT ( 'NONE',  ( -42.96289909478856117, -282.1834426611433742, -343.4306137799651424 ) ) ;
#70896=CARTESIAN_POINT ( 'NONE',  ( 28.87259822389665587, -282.9630759024261124, -236.6833557885064465 ) ) ;
#70897=CARTESIAN_POINT ( 'NONE',  ( 22.05135022558042834, -273.4265805182347435, -226.7357432167933950 ) ) ;
#70900=CARTESIAN_POINT ( 'NONE',  ( -112.0158217758180541, -279.1273359679276496, -288.5251568024719404 ) ) ;
#70904=CARTESIAN_POINT ( 'NONE',  ( -64.63248303161870467, -285.3865656027595605, -340.6147484032086368 ) ) ;
#70905=CARTESIAN_POINT ( 'NONE',  ( 19.81351785695841627, -293.3932589804636564, -316.0525511050038858 ) ) ;
#70906=CARTESIAN_POINT ( 'NONE',  ( 12.34364164194936997, -287.7296803646689227, -329.0525108734586297 ) ) ;
#70907=CARTESIAN_POINT ( 'NONE',  ( -98.17623918014778894, -283.3715890535725066, -228.1826710478582925 ) ) ;
#70908=CARTESIAN_POINT ( 'NONE',  ( -77.35434431741335004, -284.0790417985784870, -208.5401351762213267 ) ) ;
#70909=CARTESIAN_POINT ( 'NONE',  ( -76.42256932269475556, -287.8225205175797328, -333.2153913122146491 ) ) ;
#70911=CARTESIAN_POINT ( 'NONE',  ( 34.87890127943792606, -282.9298848429468762, -283.5203675050298102 ) ) ;
#70912=CARTESIAN_POINT ( 'NONE',  ( -0.9918670210656873598, -272.5344510748199127, -204.7439945824827134 ) ) ;
#70913=CARTESIAN_POINT ( 'NONE',  ( -36.55302976323596909, -284.4617733364769947, -194.1522928282763871 ) ) ;
#70914=CARTESIAN_POINT ( 'NONE',  ( -43.16067667201198788, -299.9789741420964901, -195.5353624317758374 ) ) ;
#70915=CARTESIAN_POINT ( 'NONE',  ( -26.85116024546423574, -284.1849662824337202, -195.8778696644413628 ) ) ;
#70916=CARTESIAN_POINT ( 'NONE',  ( 34.29284375403562279, -282.2924094522277301, -255.0731314231204294 ) ) ;
#70917=CARTESIAN_POINT ( 'NONE',  ( 36.31695888212765766, -289.7442375099765286, -285.3421187120097215 ) ) ;
#70922=CARTESIAN_POINT ( 'NONE',  ( 20.28556648569308507, -296.1435760537691522, -319.2325037150431513 ) ) ;
#70923=CARTESIAN_POINT ( 'NONE',  ( -65.09632711984581022, -275.4144774322957119, -340.0918235675195547 ) ) ;
#70924=CARTESIAN_POINT ( 'NONE',  ( -94.58416970613943420, -290.4461144431871844, -219.1023772910478158 ) ) ;
#70925=CARTESIAN_POINT ( 'NONE',  ( -8.941649358748334109, -293.0742662204073099, -338.4915175732525654 ) ) ;
#70926=CARTESIAN_POINT ( 'NONE',  ( -79.32294263654321753, -278.1568557582464791, -210.0384957387145164 ) ) ;
#70927=CARTESIAN_POINT ( 'NONE',  ( -67.29639256208635345, -295.7947203239685905, -202.4238560137765148 ) ) ;
#70928=CARTESIAN_POINT ( 'NONE',  ( 21.73278676675897714, -295.4761871959046289, -314.0812332294733551 ) ) ;
#70929=CARTESIAN_POINT ( 'NONE',  ( -95.99890600148557951, -299.6948066931273615, -223.6242672951989618 ) ) ;
#70930=CARTESIAN_POINT ( 'NONE',  ( -84.77021355066884212, -295.8915592484684112, -210.5845016062207264 ) ) ;
#70931=CARTESIAN_POINT ( 'NONE',  ( 6.334305210621300475, -290.0483517657721109, -329.9130267857101444 ) ) ;
#70932=CARTESIAN_POINT ( 'NONE',  ( 30.01125611929756332, -291.3308207911303498, -235.0689059052033656 ) ) ;
#70933=CARTESIAN_POINT ( 'NONE',  ( -110.9577112757685597, -292.0022508219814767, -268.4645381554518053 ) ) ;
#70935=CARTESIAN_POINT ( 'NONE',  ( -107.1587676930076185, -291.6446595430831508, -248.4515961203839538 ) ) ;
#70937=CARTESIAN_POINT ( 'NONE',  ( -113.8539525038285518, -291.7103843890140524, -274.0872357949349407 ) ) ;
#70938=CARTESIAN_POINT ( 'NONE',  ( 14.60113001986866088, -280.3454073179602801, -324.9536925428371319 ) ) ;
#70939=CARTESIAN_POINT ( 'NONE',  ( -22.74062800065226497, -292.2442654610633213, -198.8362363487564437 ) ) ;
#70940=CARTESIAN_POINT ( 'NONE',  ( 3.821971522519374442, -280.5895950612058414, -205.2247000109324802 ) ) ;
#70941=CARTESIAN_POINT ( 'NONE',  ( -13.43253302121093462, -282.4166736702749176, -343.5328066313844602 ) ) ;
#70942=CARTESIAN_POINT ( 'NONE',  ( -20.74695442014492031, -286.8384563326493435, -343.3312683061507187 ) ) ;
#70943=CARTESIAN_POINT ( 'NONE',  ( 20.65563762792238833, -279.0480263361336597, -224.0235058588398260 ) ) ;
#70944=CARTESIAN_POINT ( 'NONE',  ( -43.47659215277207068, -283.9746241947050294, -195.5605720765545925 ) ) ;
#70945=CARTESIAN_POINT ( 'NONE',  ( -28.28788035157748126, -278.6447914057597472, -194.5403293769619779 ) ) ;
#70946=CARTESIAN_POINT ( 'NONE',  ( -69.65003909050393816, -284.5570965961844649, -200.7934953595722334 ) ) ;
#70947=CARTESIAN_POINT ( 'NONE',  ( 15.55648881015009444, -275.6268389283337683, -219.7468865658700281 ) ) ;
#70949=CARTESIAN_POINT ( 'NONE',  ( -22.60053319631199997, -293.8441363279615075, -198.0483361901948456 ) ) ;
#70950=CARTESIAN_POINT ( 'NONE',  ( -32.73639169844857122, -275.5343578870714509, -194.0762026658211425 ) ) ;
#70951=CARTESIAN_POINT ( 'NONE',  ( -69.26449129827435058, -277.1507585818379198, -336.0485681243608838 ) ) ;
#70952=CARTESIAN_POINT ( 'NONE',  ( -56.19084167351235237, -291.9826410033352886, -195.6488867628638957 ) ) ;
#70953=CARTESIAN_POINT ( 'NONE',  ( -91.42051961426787443, -281.8943788855058301, -323.1322794279773234 ) ) ;
#70955=CARTESIAN_POINT ( 'NONE',  ( -33.48409333257379217, -291.1606104851200598, -197.2149591771018038 ) ) ;
#70956=CARTESIAN_POINT ( 'NONE',  ( 14.08822429628926542, -292.3298601329112216, -324.9501601104191764 ) ) ;
#70957=EDGE_LOOP ( 'NONE', ( #50571, #85894 ) ) ;
#70959=CARTESIAN_POINT ( 'NONE',  ( -57.66605211493640581, -291.2903292289551018, -200.1305009064132889 ) ) ;
#70961=CARTESIAN_POINT ( 'NONE',  ( -92.08974858914540107, -299.6948066931273047, -226.7417163044926838 ) ) ;
#70962=CARTESIAN_POINT ( 'NONE',  ( -98.04052598606990898, -296.2404562455266159, -223.3455175950362275 ) ) ;
#70963=CARTESIAN_POINT ( 'NONE',  ( 34.43121265529653385, -280.0042729836175113, -294.7923907890756254 ) ) ;
#70964=CARTESIAN_POINT ( 'NONE',  ( -87.43974517206224562, -286.6857938340589840, -212.4681002627114594 ) ) ;
#70965=CARTESIAN_POINT ( 'NONE',  ( 35.27461090180653258, -287.2868672477175664, -262.8864021414252079 ) ) ;
#70966=CARTESIAN_POINT ( 'NONE',  ( 36.04621583837688092, -277.1598641289244256, -277.0634714136897401 ) ) ;
#70967=CARTESIAN_POINT ( 'NONE',  ( -101.2932450241813314, -295.0914935827347563, -231.7632958673291910 ) ) ;
#70968=CARTESIAN_POINT ( 'NONE',  ( -111.0617634904087794, -298.4051622642763846, -263.2239262074630233 ) ) ;
#70969=CARTESIAN_POINT ( 'NONE',  ( 9.908016002244695031, -275.1789883518918600, -326.5268978601913545 ) ) ;
#70972=CARTESIAN_POINT ( 'NONE',  ( -113.7532781696036182, -296.3355659216187519, -261.0329331272471904 ) ) ;
#70973=CARTESIAN_POINT ( 'NONE',  ( 8.893081617182170717, -290.3323940235146665, -328.7020054615854860 ) ) ;
#70974=CARTESIAN_POINT ( 'NONE',  ( -43.95506239605219179, -295.9685147819440090, -195.6024511661221084 ) ) ;
#70975=CARTESIAN_POINT ( 'NONE',  ( -39.95334237696749113, -289.7371159817230932, -343.4660310767235956 ) ) ;
#70977=CARTESIAN_POINT ( 'NONE',  ( -79.77071900964088513, -278.5527743114512305, -206.3239389937831163 ) ) ;
#70978=CARTESIAN_POINT ( 'NONE',  ( -105.1676193242628727, -297.6737069820127317, -234.0133818564297314 ) ) ;
#70979=CARTESIAN_POINT ( 'NONE',  ( -69.08370068343513992, -289.7787504853539531, -201.5520164022698566 ) ) ;
#70981=CARTESIAN_POINT ( 'NONE',  ( -84.16897645924262861, -296.0092153158394126, -331.5261984271884899 ) ) ;
#70982=CARTESIAN_POINT ( 'NONE',  ( 32.64812548547408255, -293.6078836452310838, -249.3659678097900496 ) ) ;
#70986=CARTESIAN_POINT ( 'NONE',  ( -15.13535091360628293, -290.2899352147778700, -343.4203839086674179 ) ) ;
#70987=CARTESIAN_POINT ( 'NONE',  ( 13.84574458161073096, -284.9090924074130839, -334.4957818155094174 ) ) ;
#70989=CARTESIAN_POINT ( 'NONE',  ( 36.37857623291522202, -281.1776607550194171, -292.4219308133722279 ) ) ;
#70990=CARTESIAN_POINT ( 'NONE',  ( 11.11474070345475340, -284.3800312527851588, -327.4556088445825139 ) ) ;
#70991=CARTESIAN_POINT ( 'NONE',  ( 38.20576885447741233, -285.9814356807377749, -258.8202113663200521 ) ) ;
#70992=CARTESIAN_POINT ( 'NONE',  ( -89.69076770301721524, -287.8774487862178262, -323.2845468276768202 ) ) ;
#70993=CARTESIAN_POINT ( 'NONE',  ( -4.508345881559846724, -278.4845773872683026, -338.6562503927178795 ) ) ;
#70995=CARTESIAN_POINT ( 'NONE',  ( -109.9040205576796581, -278.4409636319444985, -278.7898166426994635 ) ) ;
#70996=CARTESIAN_POINT ( 'NONE',  ( -38.34693172036762121, -279.3878115182692454, -197.2536785777012653 ) ) ;
#70997=CARTESIAN_POINT ( 'NONE',  ( 22.40885946167023590, -277.2789281126348442, -318.4585332682208900 ) ) ;
#70998=CARTESIAN_POINT ( 'NONE',  ( -61.90569913442672600, -278.5348624283664662, -197.7474876212106096 ) ) ;
#70999=CARTESIAN_POINT ( 'NONE',  ( 183.1810840045989153, 262.4765370933737927, -151.7797582644170689 ) ) ;
#71000=CARTESIAN_POINT ( 'NONE',  ( -108.9514565853776418, -273.8464409009349652, -242.5585825294248821 ) ) ;
#71002=CARTESIAN_POINT ( 'NONE',  ( -29.15655736420033861, -299.5780001754430373, -193.9484034568351092 ) ) ;
#71003=CARTESIAN_POINT ( 'NONE',  ( -20.19161114001083490, -291.3376638359845856, -345.3538533559490702 ) ) ;
#71005=CARTESIAN_POINT ( 'NONE',  ( 18.06816511220410604, -289.3136505918149055, -318.4368582874723188 ) ) ;
#71006=CARTESIAN_POINT ( 'NONE',  ( -108.0932797217043912, -286.6699263575930559, -242.5017078258306071 ) ) ;
#71007=CARTESIAN_POINT ( 'NONE',  ( 30.57681734277025143, -287.2636138766055183, -297.5340165952620168 ) ) ;
#71008=CARTESIAN_POINT ( 'NONE',  ( -65.23572785461395540, -282.9147251450477825, -342.0792168366573378 ) ) ;
#71009=CARTESIAN_POINT ( 'NONE',  ( -6.415782336955198062, -278.8651154760787563, -203.3396500841393504 ) ) ;
#71010=CARTESIAN_POINT ( 'NONE',  ( -40.04218151361544642, -287.8782752587993059, -196.1750486518603225 ) ) ;
#71011=CARTESIAN_POINT ( 'NONE',  ( 25.73970730979781152, -279.5114031048926790, -232.1643675973944880 ) ) ;
#71012=CARTESIAN_POINT ( 'NONE',  ( -24.22524791666972277, -278.1964863749546453, -342.7261405411380792 ) ) ;
#71013=CARTESIAN_POINT ( 'NONE',  ( 34.68526514554316975, -275.8820380125085876, -258.0351228961662855 ) ) ;
#71014=CARTESIAN_POINT ( 'NONE',  ( -57.20282309589141079, -288.0976706260811966, -344.3993492817485844 ) ) ;
#71015=CARTESIAN_POINT ( 'NONE',  ( -65.18412495702396825, -284.2096959302913888, -341.9920363842768438 ) ) ;
#71016=CARTESIAN_POINT ( 'NONE',  ( -111.0472198917028095, -284.7668147128538862, -292.4754576098026178 ) ) ;
#71017=CARTESIAN_POINT ( 'NONE',  ( -24.06341276463702528, -283.0444876222459243, -342.1433378505650467 ) ) ;
#71020=DIRECTION ( 'NONE',  ( 1.000000000000000000, 0.000000000000000000, 0.000000000000000000 ) ) ;
#71021=CARTESIAN_POINT ( 'NONE',  ( -59.64076283008457580, -291.1983806427256809, -342.7700765517646460 ) ) ;
#71022=CARTESIAN_POINT ( 'NONE',  ( -73.18773698749311052, -290.2719188009806999, -202.7566715567104723 ) ) ;
#71023=CARTESIAN_POINT ( 'NONE',  ( -33.79202179531848316, -297.2948722605341914, -197.2001395970567046 ) ) ;
#71025=CARTESIAN_POINT ( 'NONE',  ( 0.4831257527222759807, -293.9104241770919543, -337.3284635517964034 ) ) ;
#71026=CARTESIAN_POINT ( 'NONE',  ( -108.3994899467361392, -288.7741630443317717, -290.0813334014044358 ) ) ;
#71027=CARTESIAN_POINT ( 'NONE',  ( 34.63844841391625806, -291.5671854479851959, -253.0780841330124247 ) ) ;
#71028=CARTESIAN_POINT ( 'NONE',  ( 27.38785085396388297, -289.2276159197001562, -305.0701358544159802 ) ) ;
#71029=CARTESIAN_POINT ( 'NONE',  ( -54.49178911615187815, -300.3376638359845856, -195.3683826091709363 ) ) ;
#71030=CARTESIAN_POINT ( 'NONE',  ( -74.64620179888198948, -291.5487809400572701, -335.4255076630119561 ) ) ;
#71031=CARTESIAN_POINT ( 'NONE',  ( -78.56711798594803042, -289.4987559722096080, -207.4459624674158817 ) ) ;
#71032=CARTESIAN_POINT ( 'NONE',  ( -68.14284374770194574, -293.6478781926342663, -201.9638501743547181 ) ) ;
#71033=CARTESIAN_POINT ( 'NONE',  ( -67.65599995281158385, -286.5855699896985698, -203.6943970872609952 ) ) ;
#71034=CARTESIAN_POINT ( 'NONE',  ( -7.931572173716351593, -294.4366931742251268, -201.1729190378534895 ) ) ;
#71038=CARTESIAN_POINT ( 'NONE',  ( -35.58789420918336077, -276.0539128029232643, -195.0134754155124881 ) ) ;
#71039=CARTESIAN_POINT ( 'NONE',  ( -113.2284528385501119, -295.9014665725534314, -258.2213182009091383 ) ) ;
#71040=CARTESIAN_POINT ( 'NONE',  ( 36.60060927247352680, -273.7365971362049208, -266.1027050548266857 ) ) ;
#71041=CARTESIAN_POINT ( 'NONE',  ( -73.56367644284699736, -275.6165488471139042, -335.4087207316974855 ) ) ;
#71042=CARTESIAN_POINT ( 'NONE',  ( -35.39509422559458329, -275.2821693190704195, -196.9772883050819416 ) ) ;
#71043=CARTESIAN_POINT ( 'NONE',  ( 13.58538674600394280, -273.3233641706381150, -213.3251595027922747 ) ) ;
#71044=CARTESIAN_POINT ( 'NONE',  ( -88.90184662709367558, -297.2188191018969974, -322.9391523296335436 ) ) ;
#71046=CARTESIAN_POINT ( 'NONE',  ( -79.83011133144879068, -298.2636766780665880, -210.8015961583539024 ) ) ;
#71049=CARTESIAN_POINT ( 'NONE',  ( 34.29348792924363920, -285.2697269482018214, -246.8101712888540078 ) ) ;
#71050=CARTESIAN_POINT ( 'NONE',  ( 51.66927062525243031, -299.1969939837661059, -197.3611649956296219 ) ) ;
#71051=CARTESIAN_POINT ( 'NONE',  ( 26.35736521459429227, -286.9815187556657179, -227.0775473300800229 ) ) ;
#71053=CARTESIAN_POINT ( 'NONE',  ( -102.2857046502224989, -289.6758900029295205, -311.7874237894229736 ) ) ;
#71054=CARTESIAN_POINT ( 'NONE',  ( -104.4805427056391380, -298.0804573685408627, -304.6926879629928635 ) ) ;
#71055=CARTESIAN_POINT ( 'NONE',  ( -9.839340531551428626, -292.6919539707508306, -339.9574443497089078 ) ) ;
#71056=CARTESIAN_POINT ( 'NONE',  ( -59.24630802888157177, -278.9727894298121100, -196.7109518402720028 ) ) ;
#71057=CARTESIAN_POINT ( 'NONE',  ( 39.58706461736020543, -285.0523547857347353, -270.3937649182068981 ) ) ;
#71059=CARTESIAN_POINT ( 'NONE',  ( -82.80417032364881891, -288.4849050554818746, -327.9831129786138604 ) ) ;
#71061=CARTESIAN_POINT ( 'NONE',  ( -99.00746273454316793, -287.9728612830038514, -313.0724997197551716 ) ) ;
#71062=CARTESIAN_POINT ( 'NONE',  ( -67.16106842550161105, -299.2547051593111860, -202.8399111089550217 ) ) ;
#71063=CARTESIAN_POINT ( 'NONE',  ( -39.58826171436156471, -281.4497594915775380, -193.9704268204985453 ) ) ;
#71064=CARTESIAN_POINT ( 'NONE',  ( -103.1784170829603227, -294.0854131515289396, -307.1275494892859683 ) ) ;
#71065=CARTESIAN_POINT ( 'NONE',  ( 1.101307911923784744, -282.5237073002345483, -332.4776586972570271 ) ) ;
#71066=CARTESIAN_POINT ( 'NONE',  ( -109.4367899747259969, -296.3750647719400035, -297.5540603233302477 ) ) ;
#71067=CARTESIAN_POINT ( 'NONE',  ( -69.57813917461248820, -299.1399929613908739, -204.0925752768931716 ) ) ;
#71068=CARTESIAN_POINT ( 'NONE',  ( 38.16404851057426839, -285.6831058116866302, -274.3713544293959785 ) ) ;
#71069=CARTESIAN_POINT ( 'NONE',  ( 24.61370853033482220, -282.9788861601489884, -228.0032031214378492 ) ) ;
#71070=CARTESIAN_POINT ( 'NONE',  ( -100.3750793511504611, -295.0990382903758587, -307.7464054593901324 ) ) ;
#71071=ORIENTED_EDGE ( 'NONE', *, *, #87140, .F. ) ;
#71073=CARTESIAN_POINT ( 'NONE',  ( -10.35817444959822708, -284.6783272466427093, -340.0128696143515867 ) ) ;
#71075=CARTESIAN_POINT ( 'NONE',  ( -85.33152481854864391, -287.1952119285919025, -330.4860931364850671 ) ) ;
#71076=CARTESIAN_POINT ( 'NONE',  ( 38.76564757903747704, -274.6167894020144900, -259.7861264738814384 ) ) ;
#71077=CARTESIAN_POINT ( 'NONE',  ( 32.62969052999584818, -293.1080031279846594, -249.3781517199462314 ) ) ;
#71078=CARTESIAN_POINT ( 'NONE',  ( 34.73934199120477473, -282.8711856018877597, -254.9703439682002397 ) ) ;
#71079=CARTESIAN_POINT ( 'NONE',  ( 34.36867661861910506, -277.3804864202372187, -287.8517960041486390 ) ) ;
#71080=CARTESIAN_POINT ( 'NONE',  ( -49.97805349975100597, -284.6354845063489734, -345.7732474453188161 ) ) ;
#71081=CARTESIAN_POINT ( 'NONE',  ( -97.86845138257616838, -282.7712435999849276, -311.9665010078609271 ) ) ;
#71082=CARTESIAN_POINT ( 'NONE',  ( -98.50228014096481388, -279.9620341462559736, -313.7929055038277966 ) ) ;
#71083=CARTESIAN_POINT ( 'NONE',  ( -109.1673689681241797, -273.0719936843019013, -242.4641456104056090 ) ) ;
#71084=CARTESIAN_POINT ( 'NONE',  ( 27.64768956126589927, -275.9278280799842946, -311.7564625740425868 ) ) ;
#71085=CARTESIAN_POINT ( 'NONE',  ( 25.65876316291412351, -296.0105492116871915, -310.1096752745310710 ) ) ;
#71087=CARTESIAN_POINT ( 'NONE',  ( -87.80074239612507370, -293.8875780899065262, -326.9486608867872519 ) ) ;
#71088=CARTESIAN_POINT ( 'NONE',  ( 33.89516528870262846, -274.8452658272979647, -254.0787183080210809 ) ) ;
#71089=CARTESIAN_POINT ( 'NONE',  ( -13.97578042415391586, -296.2744937728448917, -343.0023015346546345 ) ) ;
#71090=CARTESIAN_POINT ( 'NONE',  ( 25.39830413111177876, -295.3416449737861171, -314.3351323283593501 ) ) ;
#71091=CARTESIAN_POINT ( 'NONE',  ( 13.41759824623720831, -290.3405140230750590, -325.4181176257684456 ) ) ;
#71092=CARTESIAN_POINT ( 'NONE',  ( -100.7415431858061510, -276.0153548592995207, -310.2133175259565974 ) ) ;
#71093=CARTESIAN_POINT ( 'NONE',  ( -103.1181352505607833, -280.0067078608882412, -305.2147372736505986 ) ) ;
#71094=CARTESIAN_POINT ( 'NONE',  ( -109.3689979981711247, -294.3880186820214817, -289.2100530622470842 ) ) ;
#71095=CARTESIAN_POINT ( 'NONE',  ( 32.03228451635645513, -283.0178133680506107, -239.9053183300221121 ) ) ;
#71096=CARTESIAN_POINT ( 'NONE',  ( -54.81675334284438605, -284.7426530091502173, -199.1127542649804809 ) ) ;
#71097=CARTESIAN_POINT ( 'NONE',  ( -10.98649374757405184, -92.81748071270037315, -359.1663498857263903 ) ) ;
#71099=CARTESIAN_POINT ( 'NONE',  ( -107.3740255834325268, -284.4944870705180051, -249.5082399866224421 ) ) ;
#71101=CARTESIAN_POINT ( 'NONE',  ( 38.97197785513164803, -282.7336692635807935, -278.4721153531405093 ) ) ;
#71102=CARTESIAN_POINT ( 'NONE',  ( -95.50496169006194691, -284.0239253035009028, -220.4313640935382637 ) ) ;
#71103=CARTESIAN_POINT ( 'NONE',  ( -69.87360205621597231, -280.5754186639417753, -200.8162348394174614 ) ) ;
#71104=CARTESIAN_POINT ( 'NONE',  ( -69.98667028192203077, -278.9944144872179095, -339.3465316473948405 ) ) ;
#71105=CARTESIAN_POINT ( 'NONE',  ( -53.74683284575205278, -280.4984930536186880, -195.1788329381531071 ) ) ;
#71107=CARTESIAN_POINT ( 'NONE',  ( -109.1418805571601069, -299.0519495502701943, -270.3937649182068412 ) ) ;
#71108=CARTESIAN_POINT ( 'NONE',  ( 204.5908736159001080, 295.1817123384394677, -68.66699096479933928 ) ) ;
#71110=CARTESIAN_POINT ( 'NONE',  ( -33.98326286685349373, -276.0946628066722610, -195.6031797567647175 ) ) ;
#71111=CARTESIAN_POINT ( 'NONE',  ( -22.58273187492847001, -108.0340517556413147, -362.5798773164220279 ) ) ;
#71113=CARTESIAN_POINT ( 'NONE',  ( -75.32143482974849746, -277.5636852982876235, -206.0414142660602295 ) ) ;
#71114=CARTESIAN_POINT ( 'NONE',  ( -72.97857665290149498, -293.3467370114904043, -203.2346619172767817 ) ) ;
#71115=CARTESIAN_POINT ( 'NONE',  ( 22.67635874622380854, -292.3196178315226916, -228.6050766485717247 ) ) ;
#71116=CARTESIAN_POINT ( 'NONE',  ( -114.3286190704364600, -290.0490331724351449, -271.2218060457985302 ) ) ;
#71118=CARTESIAN_POINT ( 'NONE',  ( -36.30082194905342163, -293.6141135822393835, -346.7778052962706283 ) ) ;
#71119=CARTESIAN_POINT ( 'NONE',  ( -70.32184978685793908, -284.0099468332284687, -204.3261914499192358 ) ) ;
#71120=CARTESIAN_POINT ( 'NONE',  ( -33.46726754236494372, -293.9618258522103815, -196.2143852620230291 ) ) ;
#71121=CARTESIAN_POINT ( 'NONE',  ( 5.140709190119024719, -285.1177898088805591, -210.0827781962700840 ) ) ;
#71122=CARTESIAN_POINT ( 'NONE',  ( -3.378693778027990646, -283.9091123691318899, -335.5500429987772009 ) ) ;
#71124=CARTESIAN_POINT ( 'NONE',  ( -33.56297233337575392, -293.0398747076706059, -193.6894711398170443 ) ) ;
#71125=CARTESIAN_POINT ( 'NONE',  ( 24.18564823801470709, -282.5902013626234748, -309.8543107402443866 ) ) ;
#71126=CARTESIAN_POINT ( 'NONE',  ( 33.04561821504316299, -292.7355944149769584, -300.7213966613971934 ) ) ;
#71127=CARTESIAN_POINT ( 'NONE',  ( -17.75560214892808375, -289.6085933106230073, -344.6614785871051936 ) ) ;
#71128=CARTESIAN_POINT ( 'NONE',  ( -43.17137395567311131, -289.6162505669918801, -347.0784029078412800 ) ) ;
#71129=CARTESIAN_POINT ( 'NONE',  ( 19.51385372131342422, -287.0712562193587019, -224.5543500988575829 ) ) ;
#71132=CARTESIAN_POINT ( 'NONE',  ( -63.81208506680439996, -297.2540805457130659, -341.3514285980028831 ) ) ;
#71133=CARTESIAN_POINT ( 'NONE',  ( -101.1292185153662047, -295.7965146306008819, -228.0945100987094065 ) ) ;
#71134=CARTESIAN_POINT ( 'NONE',  ( -103.3482622026562012, -277.1816553580022742, -302.2045485854078493 ) ) ;
#71136=CARTESIAN_POINT ( 'NONE',  ( -73.91008298179929170, -273.0878264126634463, -202.6093528009212150 ) ) ;
#71137=CARTESIAN_POINT ( 'NONE',  ( -67.59740104981793252, -293.9363353241926120, -337.5709406013941702 ) ) ;
#71138=CARTESIAN_POINT ( 'NONE',  ( 36.65556519529913260, -277.2922338544670993, -268.8188029703112534 ) ) ;
#71139=CARTESIAN_POINT ( 'NONE',  ( -111.5760183017738854, -270.7279678523428856, -267.5675363796792112 ) ) ;
#71140=CARTESIAN_POINT ( 'NONE',  ( -104.2925540072696293, -297.3527687345801951, -300.5637557906787265 ) ) ;
#71141=CARTESIAN_POINT ( 'NONE',  ( -107.1594597061730383, -297.3346759082611470, -292.8794707580600516 ) ) ;
#71143=CARTESIAN_POINT ( 'NONE',  ( -36.26509739655411835, -296.6390247100388819, -346.5664821968878755 ) ) ;
#71144=CARTESIAN_POINT ( 'NONE',  ( -111.8392290246089402, -294.4188869387747900, -280.7506060141661237 ) ) ;
#71145=CARTESIAN_POINT ( 'NONE',  ( -111.6647335822579095, -273.6019179559034455, -250.6574968307645577 ) ) ;
#71146=CARTESIAN_POINT ( 'NONE',  ( -102.1707620524067295, -288.6545596536325888, -305.2911486288720653 ) ) ;
#71147=CARTESIAN_POINT ( 'NONE',  ( -72.87722998788049722, -275.5819331601612134, -204.2560866829686574 ) ) ;
#71148=CARTESIAN_POINT ( 'NONE',  ( -109.1114665446813206, -273.3976083949872873, -242.4903039726218879 ) ) ;
#71149=CARTESIAN_POINT ( 'NONE',  ( -109.2974171359836788, -297.0493369894550710, -257.9328326343158437 ) ) ;
#71150=CARTESIAN_POINT ( 'NONE',  ( -53.43434310871793969, -281.8267582749264761, -196.6909084885670040 ) ) ;
#71151=CARTESIAN_POINT ( 'NONE',  ( 8.266075918669939071, -279.3460740564684670, -208.8686381655618050 ) ) ;
#71153=CARTESIAN_POINT ( 'NONE',  ( 21.52662368116387626, -281.5678167806487409, -319.8367002313106013 ) ) ;
#71154=CARTESIAN_POINT ( 'NONE',  ( 37.13794643748232716, -275.1405084822180243, -289.4947280554013105 ) ) ;
#71155=CARTESIAN_POINT ( 'NONE',  ( 12.48460853774552604, -279.1329237015384024, -212.7088901135653600 ) ) ;
#71156=CARTESIAN_POINT ( 'NONE',  ( -93.57296505719520496, -277.2443382476839702, -220.4805278424888684 ) ) ;
#71158=CARTESIAN_POINT ( 'NONE',  ( -87.72359660053737684, -271.9067572238526509, -216.6533259070059216 ) ) ;
#71159=CARTESIAN_POINT ( 'NONE',  ( 35.98171872038178520, -277.7555091975439154, -286.1901677788409870 ) ) ;
#71162=CARTESIAN_POINT ( 'NONE',  ( -100.6923248960869444, -295.3516191973229184, -228.3770683574962845 ) ) ;
#71163=CARTESIAN_POINT ( 'NONE',  ( 0.8878766968512699087, -290.5791947935748567, -205.3637653945487500 ) ) ;
#71164=CARTESIAN_POINT ( 'NONE',  ( -95.66091589783415827, -291.2312609012022335, -220.0630462660494970 ) ) ;
#71166=CARTESIAN_POINT ( 'NONE',  ( 2.550636152687149938, -278.5192513579186198, -334.1297771630124203 ) ) ;
#71167=CARTESIAN_POINT ( 'NONE',  ( -66.56969732517289629, -271.6691758511835815, -201.2906841448159696 ) ) ;
#71169=CARTESIAN_POINT ( 'NONE',  ( -55.33512605364504822, -285.2020442254257659, -343.7474301847148013 ) ) ;
#71171=CARTESIAN_POINT ( 'NONE',  ( -91.23782066981317485, -281.8177728978624259, -322.5895926092773038 ) ) ;
#71173=CARTESIAN_POINT ( 'NONE',  ( 19.12882268324476343, -293.0084871546870886, -317.2461961995161346 ) ) ;
#71174=CARTESIAN_POINT ( 'NONE',  ( 20.49216839403380419, -285.0444886364653598, -223.7994926256597807 ) ) ;
#71176=CARTESIAN_POINT ( 'NONE',  ( -45.32835983327135665, -293.1530363356147291, -344.9865251391520928 ) ) ;
#71177=CARTESIAN_POINT ( 'NONE',  ( -111.6798620076071984, -283.2493622608496366, -253.1406230943017874 ) ) ;
#71178=CARTESIAN_POINT ( 'NONE',  ( -72.52888815605126638, -281.1782274276820317, -205.4896896412770104 ) ) ;
#71179=CARTESIAN_POINT ( 'NONE',  ( -63.08252603085015409, -286.9292845945221302, -198.2125310249039956 ) ) ;
#71180=CARTESIAN_POINT ( 'NONE',  ( 22.95705254234390935, -279.1668047485427451, -224.1009697138881052 ) ) ;
#71181=CARTESIAN_POINT ( 'NONE',  ( 33.99600683975054238, -287.3478169724168652, -254.8713934991565395 ) ) ;
#71182=CARTESIAN_POINT ( 'NONE',  ( -107.6744403733134305, -279.6909400585233811, -292.1806430036223787 ) ) ;
#71183=CARTESIAN_POINT ( 'NONE',  ( -87.64906402838282418, -280.1309426497939512, -217.1707527470145749 ) ) ;
#71184=CARTESIAN_POINT ( 'NONE',  ( -96.30940390701977094, -287.1738436537719394, -223.4439919097640370 ) ) ;
#71187=CARTESIAN_POINT ( 'NONE',  ( -89.60674544234061045, -297.1730543878309732, -213.7436443667388914 ) ) ;
#71189=CARTESIAN_POINT ( 'NONE',  ( 36.59295671128113270, -289.6657690718142248, -280.7263723183225466 ) ) ;
#71191=CARTESIAN_POINT ( 'NONE',  ( 40.65961533371913106, -284.2662352645559167, -288.1317622949166548 ) ) ;
#71193=CARTESIAN_POINT ( 'NONE',  ( 32.03159489696659534, -273.1734711455305842, -241.2891532907173371 ) ) ;
#71194=CARTESIAN_POINT ( 'NONE',  ( 32.59827851968617551, -291.5625646331923235, -240.1147991936883557 ) ) ;
#71195=CARTESIAN_POINT ( 'NONE',  ( -49.95838822131641876, -297.3944571262421732, -198.3971851894851284 ) ) ;
#71196=CARTESIAN_POINT ( 'NONE',  ( 22.54379778067782070, -288.4765996302595568, -227.3282294425881958 ) ) ;
#71197=CARTESIAN_POINT ( 'NONE',  ( 35.56141040672193299, -283.1461264425809077, -257.5896462922316346 ) ) ;
#71198=CARTESIAN_POINT ( 'NONE',  ( -104.6284536667436669, -291.5056410137439684, -306.5702202861667161 ) ) ;
#71199=CARTESIAN_POINT ( 'NONE',  ( -98.62400573995364539, -291.2537730180500830, -316.1842751939321943 ) ) ;
#71200=CARTESIAN_POINT ( 'NONE',  ( -110.3172948394246333, -286.7751970360466771, -252.9978314765042740 ) ) ;
#71201=CARTESIAN_POINT ( 'NONE',  ( -59.66298242062732271, -277.5001923794367826, -344.0548108015921116 ) ) ;
#71203=CARTESIAN_POINT ( 'NONE',  ( -34.92564695030645083, -293.1018725119407691, -345.8824850763513155 ) ) ;
#71204=CARTESIAN_POINT ( 'NONE',  ( 39.41187872584406193, -281.3084916093469587, -264.2057839050835923 ) ) ;
#71205=CARTESIAN_POINT ( 'NONE',  ( 19.93705533788776663, -276.7544095775580217, -223.1381399350777883 ) ) ;
#71206=CARTESIAN_POINT ( 'NONE',  ( -82.08285599513421005, -280.1948066931273615, -326.5171145203363494 ) ) ;
#71207=CARTESIAN_POINT ( 'NONE',  ( 38.61848655886215909, -273.7665885328542572, -268.3551145334367334 ) ) ;
#71209=CARTESIAN_POINT ( 'NONE',  ( 0.4371355078812793060, -280.0775711935852996, -207.7665775492066302 ) ) ;
#71210=CARTESIAN_POINT ( 'NONE',  ( -91.03969113989829509, -278.9990767769909326, -325.0662779953688073 ) ) ;
#71211=CARTESIAN_POINT ( 'NONE',  ( -63.49778399579081167, -275.0192065503160848, -201.6663645440007429 ) ) ;
#71212=CARTESIAN_POINT ( 'NONE',  ( -67.08678917969932343, -284.7303750366101553, -199.5935414335779967 ) ) ;
#71213=CARTESIAN_POINT ( 'NONE',  ( -109.9281863996342423, -292.1232755092998445, -284.8887651978565714 ) ) ;
#71214=CARTESIAN_POINT ( 'NONE',  ( -31.34357104310445763, -275.7268071014981956, -194.3844119261464130 ) ) ;
#71215=CARTESIAN_POINT ( 'NONE',  ( -83.29732934001472699, -274.7527717440063952, -209.1279932916463622 ) ) ;
#71217=CARTESIAN_POINT ( 'NONE',  ( -112.0711609299673910, -298.5015950478284594, -274.3027054896107302 ) ) ;
#71218=CARTESIAN_POINT ( 'NONE',  ( -109.1583620544447939, -282.2800102413123682, -291.4401240812232459 ) ) ;
#71219=CARTESIAN_POINT ( 'NONE',  ( -114.1664693979008263, -290.2797717242427211, -265.4929439832420712 ) ) ;
#71220=CARTESIAN_POINT ( 'NONE',  ( 4.025136767110162772, -274.5119387591219606, -332.4950990723469317 ) ) ;
#71221=CARTESIAN_POINT ( 'NONE',  ( 9.304787896971838279, -288.2812600259862279, -210.1071092500549753 ) ) ;
#71222=CARTESIAN_POINT ( 'NONE',  ( -110.5534919926727184, -289.5336725926654822, -265.7023306903804496 ) ) ;
#71224=CARTESIAN_POINT ( 'NONE',  ( -104.6456110209736181, -288.6555553013054691, -306.5383189512274384 ) ) ;
#71225=CARTESIAN_POINT ( 'NONE',  ( -108.4470887267320052, -290.4387262007506365, -253.6900082406413048 ) ) ;
#71227=CARTESIAN_POINT ( 'NONE',  ( 39.39339127847529198, -288.6465345582640225, -271.5327885895955546 ) ) ;
#71228=CARTESIAN_POINT ( 'NONE',  ( -94.81012767768720551, -279.5206241622084917, -225.2913814188073047 ) ) ;
#71229=ADVANCED_FACE ( 'NONE', ( #55777 ), #92705, .T. ) ;
#71230=CARTESIAN_POINT ( 'NONE',  ( -84.00804977312975552, -294.5964901115760313, -331.2864785464611828 ) ) ;
#71231=CARTESIAN_POINT ( 'NONE',  ( -86.03141575334062452, -284.3584066722862644, -329.8810673995528191 ) ) ;
#71232=CARTESIAN_POINT ( 'NONE',  ( -36.56990796445238345, -286.3948696416265989, -193.3730956640566774 ) ) ;
#71233=CARTESIAN_POINT ( 'NONE',  ( 22.60455508182450757, -282.4664161788334127, -312.0568488564973109 ) ) ;
#71234=CARTESIAN_POINT ( 'NONE',  ( -48.27666066358466423, -154.8625263976673807, -365.1983507399203290 ) ) ;
#71235=CARTESIAN_POINT ( 'NONE',  ( 198.2119960356330068, 289.1949541700149098, -97.17456560034590041 ) ) ;
#71236=CARTESIAN_POINT ( 'NONE',  ( 137.5249753115113833, 179.0922514384929514, -238.4867443683607462 ) ) ;
#71237=CARTESIAN_POINT ( 'NONE',  ( -24.55819114827195904, -273.4165044668659448, -198.2734257282029660 ) ) ;
#71238=CARTESIAN_POINT ( 'NONE',  ( -19.18181074326775715, -273.2115671961610133, -199.2842135568791662 ) ) ;
#71239=CARTESIAN_POINT ( 'NONE',  ( -65.58674650670324979, -294.9193915616468189, -341.9416917330253796 ) ) ;
#71240=CARTESIAN_POINT ( 'NONE',  ( 180.4165302251282981, 251.0051037841290054, -164.4917810413223549 ) ) ;
#71241=CARTESIAN_POINT ( 'NONE',  ( -35.51864135670681577, -272.7593795388713716, -193.8629445613833013 ) ) ;
#71242=CARTESIAN_POINT ( 'NONE',  ( -106.9725360597648205, -298.7517750038622353, -244.4753471587631566 ) ) ;
#71243=CARTESIAN_POINT ( 'NONE',  ( -77.43566305231442470, -292.5798602431752897, -208.9876692430420064 ) ) ;
#71245=CARTESIAN_POINT ( 'NONE',  ( -105.7425838429125378, -297.0419842968203170, -305.3226787405124583 ) ) ;
#71247=CARTESIAN_POINT ( 'NONE',  ( -34.56939098001380017, -289.5088680095021232, -343.4196635109688600 ) ) ;
#71248=CARTESIAN_POINT ( 'NONE',  ( -3.291124993926298981, -295.4168373338897027, -339.2575993944697643 ) ) ;
#71249=CARTESIAN_POINT ( 'NONE',  ( -77.04509521186594156, -296.0611028403902765, -336.3258073262312564 ) ) ;
#71250=CARTESIAN_POINT ( 'NONE',  ( 26.23351112299397769, -293.2265036997508787, -234.3804449044959881 ) ) ;
#71252=CARTESIAN_POINT ( 'NONE',  ( 29.28508072594790335, -277.9429568179117496, -306.1113322268128059 ) ) ;
#71255=CARTESIAN_POINT ( 'NONE',  ( -114.1490536736508403, -278.1160007762876489, -265.8714248523405672 ) ) ;
#71256=CARTESIAN_POINT ( 'NONE',  ( 35.58941446579279244, -276.5810874108776716, -277.0290240886006927 ) ) ;
#71257=CARTESIAN_POINT ( 'NONE',  ( -1.795634698020047493, -276.2766762443887387, -203.2012248316537182 ) ) ;
#71259=CARTESIAN_POINT ( 'NONE',  ( 19.56129288270044242, -274.2546427920289034, -319.7816128438179248 ) ) ;
#71260=CARTESIAN_POINT ( 'NONE',  ( -41.88295005433539586, -298.6448310457113280, -197.4003770499783457 ) ) ;
#71261=CARTESIAN_POINT ( 'NONE',  ( -108.1748622820848880, -294.8652590384936047, -290.3120091230533149 ) ) ;
#71263=CARTESIAN_POINT ( 'NONE',  ( -114.0172163562985617, -278.9572510882937308, -277.3317464269327388 ) ) ;
#71264=CARTESIAN_POINT ( 'NONE',  ( -39.15563525293699598, -277.2422278009347565, -343.3385778170336948 ) ) ;
#71265=CARTESIAN_POINT ( 'NONE',  ( -36.55358155725070901, -284.7466815336893546, -193.8453704683005867 ) ) ;
#71266=CARTESIAN_POINT ( 'NONE',  ( -88.38255267908760970, -299.3395460214596824, -215.1103382808467472 ) ) ;
#71267=CARTESIAN_POINT ( 'NONE',  ( 82.68068823132855982, -297.0576872996817883, -195.5766972444398277 ) ) ;
#71268=CARTESIAN_POINT ( 'NONE',  ( -3.300329454211856195, -287.7880372195716632, -335.1766745257123148 ) ) ;
#71270=CARTESIAN_POINT ( 'NONE',  ( -13.96789683373837043, -278.5993066953135440, -200.0812993349136093 ) ) ;
#71271=CARTESIAN_POINT ( 'NONE',  ( -30.18717691561256444, -278.7190183630609113, -197.0697410520693609 ) ) ;
#71272=CARTESIAN_POINT ( 'NONE',  ( -80.26349666223615031, -287.4714558594855589, -208.7946902293803362 ) ) ;
#71273=CARTESIAN_POINT ( 'NONE',  ( -37.79690201333477262, -278.2630203141016523, -343.7693015118818494 ) ) ;
#71275=CARTESIAN_POINT ( 'NONE',  ( -108.7917012335690998, -276.4592604694012721, -296.3777157158555724 ) ) ;
#71276=CARTESIAN_POINT ( 'NONE',  ( 23.87433217131118823, -275.6506605213479020, -230.4050163498186521 ) ) ;
#71277=CARTESIAN_POINT ( 'NONE',  ( 36.08038257627535472, -283.7593415663213250, -286.5211524010406947 ) ) ;
#71278=DIRECTION ( 'NONE',  ( 0.000000000000000000, 0.000000000000000000, -1.000000000000000000 ) ) ;
#71279=CARTESIAN_POINT ( 'NONE',  ( 38.19986181628766531, -289.4510330571735608, -268.6918024929133821 ) ) ;
#71280=CARTESIAN_POINT ( 'NONE',  ( -37.21641030581353249, -290.0535995824776592, -195.3486460966812501 ) ) ;
#71282=CARTESIAN_POINT ( 'NONE',  ( 17.66572841636178737, -273.5445591991725109, -221.5473438095443726 ) ) ;
#71283=CARTESIAN_POINT ( 'NONE',  ( 31.00203996097383197, -291.3075500401632212, -241.2467744551517228 ) ) ;
#71284=CARTESIAN_POINT ( 'NONE',  ( 84.09003387609358526, 83.72762891241104910, -302.5758382668069544 ) ) ;
#71286=CARTESIAN_POINT ( 'NONE',  ( -37.51958215299946175, -287.5341899270762269, -346.6805335928127647 ) ) ;
#71287=CARTESIAN_POINT ( 'NONE',  ( -92.24673890178284807, -285.4539155900227456, -319.6941935321918891 ) ) ;
#71288=CARTESIAN_POINT ( 'NONE',  ( 9.207898403482005278, -284.9215312258402832, -210.3019064671752858 ) ) ;
#71289=CARTESIAN_POINT ( 'NONE',  ( -98.00789117072753243, -285.4011671194150495, -312.1030888942941601 ) ) ;
#71291=CARTESIAN_POINT ( 'NONE',  ( -42.93508183178217763, -283.9272458198304889, -343.3586650328691121 ) ) ;
#71292=CARTESIAN_POINT ( 'NONE',  ( -111.0368374297748488, -292.7338024474436224, -254.5701208483027642 ) ) ;
#71293=CARTESIAN_POINT ( 'NONE',  ( 32.39416771235466541, -273.2534646911319669, -241.1359645824260554 ) ) ;
#71294=CARTESIAN_POINT ( 'NONE',  ( -41.19595950263610007, -274.3383013758099764, -193.4265667472966186 ) ) ;
#71295=CARTESIAN_POINT ( 'NONE',  ( -112.2354221227958107, -288.7644722007285054, -259.9667589313752956 ) ) ;
#71296=CARTESIAN_POINT ( 'NONE',  ( -28.60103679366061868, -276.9443428542415973, -346.9169861407146414 ) ) ;
#71297=CARTESIAN_POINT ( 'NONE',  ( 13.49307001322679866, -296.3166846005143498, -325.0915939867428506 ) ) ;
#71299=CARTESIAN_POINT ( 'NONE',  ( -95.33595429735161986, -283.8690164008716010, -225.1974727807570389 ) ) ;
#71300=CARTESIAN_POINT ( 'NONE',  ( -72.79708432511026217, -277.5824163068654116, -204.2563438829853908 ) ) ;
#71302=CARTESIAN_POINT ( 'NONE',  ( -64.63385711970310865, -272.1821061786632185, -199.0880557362332866 ) ) ;
#71303=CARTESIAN_POINT ( 'NONE',  ( -93.68989878019139894, -277.2412800259394885, -316.9508224767259321 ) ) ;
#71304=CARTESIAN_POINT ( 'NONE',  ( 12.84104884053895468, -295.8569884145592823, -324.3977272391306883 ) ) ;
#71305=CARTESIAN_POINT ( 'NONE',  ( 18.94268244307061266, -279.7600730235698734, -218.2692684433834529 ) ) ;
#71306=CARTESIAN_POINT ( 'NONE',  ( 3.958929688774724731, -295.4217909888135978, -330.8397623485831218 ) ) ;
#71307=CARTESIAN_POINT ( 'NONE',  ( -22.17880000799752693, -296.1770039131457111, -345.3503487520475801 ) ) ;
#71308=CARTESIAN_POINT ( 'NONE',  ( -97.85833484114162673, -272.7877700927374462, -229.4074339833789509 ) ) ;
#71309=CARTESIAN_POINT ( 'NONE',  ( -95.86716431267517180, -293.1976446539002836, -223.4389891019135064 ) ) ;
#71310=CARTESIAN_POINT ( 'NONE',  ( -114.3407763534793133, -284.7235490238601869, -269.9839377611181703 ) ) ;
#71311=CARTESIAN_POINT ( 'NONE',  ( -63.11429437396755304, -271.8595950360511324, -199.1145119892237858 ) ) ;
#71312=CARTESIAN_POINT ( 'NONE',  ( 39.09029681861581196, -287.5075871118602322, -280.1252899188548326 ) ) ;
#71313=CARTESIAN_POINT ( 'NONE',  ( -52.17841053344522351, -281.8413174996396720, -197.1527759572261971 ) ) ;
#71314=CARTESIAN_POINT ( 'NONE',  ( -70.07688052730672723, -284.6687166075377036, -204.8351735597303218 ) ) ;
#71315=CARTESIAN_POINT ( 'NONE',  ( -31.99545433121289761, -286.9846679685006166, -345.2215219216343485 ) ) ;
#71316=CARTESIAN_POINT ( 'NONE',  ( -101.2450674239233592, -254.4445186991787295, -323.9438275447045612 ) ) ;
#71317=CARTESIAN_POINT ( 'NONE',  ( -25.12536402201791930, -285.7196489527982521, -198.2768005689917175 ) ) ;
#71319=CARTESIAN_POINT ( 'NONE',  ( -38.71627898499669129, -284.0102451876064720, -347.1135169473235464 ) ) ;
#71320=CARTESIAN_POINT ( 'NONE',  ( -112.6395549005616914, -289.4227131745509496, -285.3627656624889255 ) ) ;
#71321=CARTESIAN_POINT ( 'NONE',  ( -74.63438397662177692, -281.1645436758938672, -203.9104133411500186 ) ) ;
#71322=CARTESIAN_POINT ( 'NONE',  ( -99.24084800811483831, -279.2666289216291489, -315.3477493140125603 ) ) ;
#71323=CARTESIAN_POINT ( 'NONE',  ( 19.67734598586952899, -280.7414879347180090, -224.7779151025930275 ) ) ;
#71324=CARTESIAN_POINT ( 'NONE',  ( 37.64196114685309169, -277.5322144740228509, -268.7954911116262338 ) ) ;
#71325=CARTESIAN_POINT ( 'NONE',  ( 21.36765032522750829, -294.2237324663467462, -320.1829221384771245 ) ) ;
#71326=CARTESIAN_POINT ( 'NONE',  ( -15.39151440710578100, -286.7868564360038590, -341.7596160424234881 ) ) ;
#71327=AXIS2_PLACEMENT_3D ( 'NONE', #31559, #73717, #38169 ) ;
#71328=CARTESIAN_POINT ( 'NONE',  ( -110.6936164896955859, -295.4581172883108593, -271.4540624634458936 ) ) ;
#71331=CARTESIAN_POINT ( 'NONE',  ( 22.99316106881965638, -284.0706602695782976, -313.9836256508349948 ) ) ;
#71332=CARTESIAN_POINT ( 'NONE',  ( -66.06536231592032493, -295.1054502257089212, -337.4956003098182578 ) ) ;
#71333=CARTESIAN_POINT ( 'NONE',  ( 35.15587675956225411, -294.3134460322865493, -245.1885792623658631 ) ) ;
#71334=CARTESIAN_POINT ( 'NONE',  ( -56.33740688475722891, -283.9548921245145152, -340.9518807824663895 ) ) ;
#71335=CARTESIAN_POINT ( 'NONE',  ( -31.26669625731216939, -273.1858367891194348, -193.8239296604105277 ) ) ;
#71336=CARTESIAN_POINT ( 'NONE',  ( -89.41635397459970136, -290.4144857261113657, -326.9432990389424276 ) ) ;
#71337=CARTESIAN_POINT ( 'NONE',  ( -89.60354244762366704, -281.9186581479480651, -325.2874780045280545 ) ) ;
#71338=CARTESIAN_POINT ( 'NONE',  ( -103.7780316256559274, -290.3780176433012912, -309.3504474542032199 ) ) ;
#71339=CARTESIAN_POINT ( 'NONE',  ( 24.25846200230541072, -288.4274304494380772, -309.5721816287082220 ) ) ;
#71342=CARTESIAN_POINT ( 'NONE',  ( 167.6084280626006944, 229.7879449464658421, -189.9070988384416410 ) ) ;
#71343=CARTESIAN_POINT ( 'NONE',  ( -54.42813229853333468, -277.3380690714490697, -195.3538533559490702 ) ) ;
#71345=CARTESIAN_POINT ( 'NONE',  ( -11.62187183220122044, -279.3153257988083169, -201.6582016399473503 ) ) ;
#71346=CARTESIAN_POINT ( 'NONE',  ( 9.500835673342779231, -274.3434189508841428, -209.2749400768466614 ) ) ;
#71347=CARTESIAN_POINT ( 'NONE',  ( -39.17784308802448834, -279.0754116944869452, -345.1719260844724317 ) ) ;
#71348=CARTESIAN_POINT ( 'NONE',  ( 186.5835289679585571, 260.6838375247356225, -151.8520429253792088 ) ) ;
#71349=CARTESIAN_POINT ( 'NONE',  ( -113.1302542624162726, -277.2545904217303132, -260.2278703014147823 ) ) ;
#71350=CARTESIAN_POINT ( 'NONE',  ( -70.97818951900022455, -281.5182739647821109, -337.0119904641340440 ) ) ;
#71351=CARTESIAN_POINT ( 'NONE',  ( -103.7068162096752673, -297.8248444825496222, -307.4773476484015191 ) ) ;
#71352=CARTESIAN_POINT ( 'NONE',  ( -0.7216792812276195956, -295.0443016268835663, -333.6403975773210959 ) ) ;
#71354=CARTESIAN_POINT ( 'NONE',  ( -102.0854682574641430, -288.7646402153769145, -305.2467552421152277 ) ) ;
#71355=CARTESIAN_POINT ( 'NONE',  ( 1.137220292409873545, -275.2032020103217178, -203.7674380173210409 ) ) ;
#71356=CARTESIAN_POINT ( 'NONE',  ( -107.9400821963975687, -272.7996867053294636, -251.5966473179044840 ) ) ;
#71363=CARTESIAN_POINT ( 'NONE',  ( -67.44574272812705829, -280.7274322649572582, -203.5045570478806098 ) ) ;
#71364=CARTESIAN_POINT ( 'NONE',  ( -64.40269168991542870, -281.4640483969555476, -199.3008551396109738 ) ) ;
#71365=CARTESIAN_POINT ( 'NONE',  ( -92.74496407832654654, -282.9305115132227684, -318.2747440884989487 ) ) ;
#71366=CARTESIAN_POINT ( 'NONE',  ( -34.28580327928959548, -281.9513627311629875, -196.1760830298977680 ) ) ;
#71367=CARTESIAN_POINT ( 'NONE',  ( 17.94266555293387100, -274.7215094061202763, -319.1074171479883717 ) ) ;
#71370=CARTESIAN_POINT ( 'NONE',  ( -96.01924808991735460, -278.6849791212837317, -319.9909397655279690 ) ) ;
#71374=CARTESIAN_POINT ( 'NONE',  ( -95.87840379837734872, -285.8814319001881472, -317.8351667553786228 ) ) ;
#71375=CARTESIAN_POINT ( 'NONE',  ( 18.95080791339541548, -293.4106652269962865, -317.0917852779367649 ) ) ;
#71376=CARTESIAN_POINT ( 'NONE',  ( 5.493655457592956814, -287.8371250870607696, -334.2238230474468992 ) ) ;
#71377=CARTESIAN_POINT ( 'NONE',  ( -110.6122710711097739, -282.9280929730704202, -259.9017945200786812 ) ) ;
#71378=CARTESIAN_POINT ( 'NONE',  ( -86.10311347677664173, -283.9353757169868118, -215.1776970751005820 ) ) ;
#71379=CARTESIAN_POINT ( 'NONE',  ( -85.35925401383246935, -287.9658603153652621, -326.7518551005912855 ) ) ;
#71380=CARTESIAN_POINT ( 'NONE',  ( 10.17738979605122829, -283.5850744603056341, -326.3660279873531636 ) ) ;
#71381=CARTESIAN_POINT ( 'NONE',  ( -11.02489460564906487, -272.3948899110692423, -200.0746247869440708 ) ) ;
#71383=CARTESIAN_POINT ( 'NONE',  ( -111.4459895149638413, -282.7270380410681696, -288.1645036816406105 ) ) ;
#71384=CARTESIAN_POINT ( 'NONE',  ( -108.4414061454866243, -298.2436910454931080, -294.2322815991927882 ) ) ;
#71385=CARTESIAN_POINT ( 'NONE',  ( -35.17493780986814755, -284.0791100049262923, -195.2128528951598980 ) ) ;
#71387=CARTESIAN_POINT ( 'NONE',  ( -109.5159295249515452, -279.3291025618385675, -282.8564870290426825 ) ) ;
#71388=CARTESIAN_POINT ( 'NONE',  ( 24.36169394290485712, -290.1344191215795263, -313.3774366260588522 ) ) ;
#71391=CARTESIAN_POINT ( 'NONE',  ( 37.39589411695873622, -295.6139983819052759, -281.4789507191275106 ) ) ;
#71393=CARTESIAN_POINT ( 'NONE',  ( -97.71778290525287503, -275.9448053321831367, -314.8768026644906399 ) ) ;
#71394=CARTESIAN_POINT ( 'NONE',  ( -114.0905082423682160, -289.7027993248532312, -274.0731623080545774 ) ) ;
#71395=CARTESIAN_POINT ( 'NONE',  ( 27.85536805538228222, -292.4192895141347890, -305.0503552548572657 ) ) ;
#71396=CARTESIAN_POINT ( 'NONE',  ( -68.71874049333912637, -278.3156349909451706, -203.9026736917828373 ) ) ;
#71397=CARTESIAN_POINT ( 'NONE',  ( -99.02293217888494326, -271.2011532360954220, -228.5949914414455861 ) ) ;
#71398=CARTESIAN_POINT ( 'NONE',  ( -97.17252897901096276, -292.4606161553429047, -227.5957976191457988 ) ) ;
#71399=CARTESIAN_POINT ( 'NONE',  ( 35.78497577281001440, -284.2662352645559167, -287.0191576251351080 ) ) ;
#71400=CARTESIAN_POINT ( 'NONE',  ( -70.52403406787870210, -293.9615079234934569, -339.0896929176657864 ) ) ;
#71401=CARTESIAN_POINT ( 'NONE',  ( -97.99490420138005220, -291.5725689488497778, -312.4264946828913025 ) ) ;
#71402=CARTESIAN_POINT ( 'NONE',  ( 31.28061286755202985, -291.3667596246654625, -237.6051557016747608 ) ) ;
#71403=CARTESIAN_POINT ( 'NONE',  ( -106.5808803370746745, -291.6481052360687158, -295.2872255897697187 ) ) ;
#71406=CARTESIAN_POINT ( 'NONE',  ( -108.8182862165075449, -291.1487983392687511, -286.0301920086504879 ) ) ;
#71408=CARTESIAN_POINT ( 'NONE',  ( -112.4755151888254119, -291.5686938336393155, -285.3579968711046035 ) ) ;
#71409=CARTESIAN_POINT ( 'NONE',  ( 37.99729989076480763, -279.5312607891003154, -267.1530959016654947 ) ) ;
#71410=CARTESIAN_POINT ( 'NONE',  ( -1.256675880218204533, -292.5451282510546207, -206.8890109921680676 ) ) ;
#71411=CARTESIAN_POINT ( 'NONE',  ( 32.02146675891162886, -281.1218690377303346, -236.8056672198304113 ) ) ;
#71412=CARTESIAN_POINT ( 'NONE',  ( 32.37143901423192460, -281.6384311189004848, -303.1336246565859369 ) ) ;
#71413=CARTESIAN_POINT ( 'NONE',  ( -3.674546666726771882, -284.4963017798824580, -203.3422890575180020 ) ) ;
#71414=CARTESIAN_POINT ( 'NONE',  ( -0.6619558416067039541, -280.6988714198547541, -334.9015071981390292 ) ) ;
#71415=CARTESIAN_POINT ( 'NONE',  ( -32.41176746138095410, -284.1141308810636588, -195.5104930882962719 ) ) ;
#71416=CARTESIAN_POINT ( 'NONE',  ( 23.20906207924225484, -279.4067851733914267, -223.9036488897866093 ) ) ;
#71417=CARTESIAN_POINT ( 'NONE',  ( 7.374898859765222525, -285.5660353292421973, -207.9906607808457295 ) ) ;
#71418=CARTESIAN_POINT ( 'NONE',  ( 5.262497132025202085, -275.4476596105712360, -210.8217563982392164 ) ) ;
#71420=CARTESIAN_POINT ( 'NONE',  ( -52.55436324774615997, -293.4543107966954949, -198.0935823730684433 ) ) ;
#71421=CARTESIAN_POINT ( 'NONE',  ( 29.42378339552801592, -276.4907415538869486, -233.0908697664995657 ) ) ;
#71422=CARTESIAN_POINT ( 'NONE',  ( -108.5078298940611177, -278.0024587740880975, -286.7710388224467124 ) ) ;
#71423=CARTESIAN_POINT ( 'NONE',  ( -114.3901020438053848, -290.7079543581995722, -271.2308759439659980 ) ) ;
#71424=CARTESIAN_POINT ( 'NONE',  ( 37.75452565523089277, -279.5196107165972421, -261.5427661957741634 ) ) ;
#71425=CARTESIAN_POINT ( 'NONE',  ( -56.18673276623513857, -291.6493345696363804, -195.6478503356330236 ) ) ;
#71426=CARTESIAN_POINT ( 'NONE',  ( -36.19044573032927303, -291.1256462782791345, -197.1223557603116774 ) ) ;
#71427=CARTESIAN_POINT ( 'NONE',  ( 24.06218792717892541, -292.1369262873832895, -313.4481604880837722 ) ) ;
#71430=CARTESIAN_POINT ( 'NONE',  ( 8.892626217268210453, -292.2136587735435000, -213.7236311021974586 ) ) ;
#71432=CARTESIAN_POINT ( 'NONE',  ( -6.998514795304330072, -274.1237833571632905, -333.4427485647536855 ) ) ;
#71433=CARTESIAN_POINT ( 'NONE',  ( -101.4384328853939650, -295.0526783255725718, -312.6997769162933309 ) ) ;
#71434=CARTESIAN_POINT ( 'NONE',  ( -110.4597285074341926, -286.1539619006878183, -247.6648574772274287 ) ) ;
#71435=CARTESIAN_POINT ( 'NONE',  ( -25.13973092812124932, -286.0452636887555400, -198.3368251598397478 ) ) ;
#71436=CARTESIAN_POINT ( 'NONE',  ( 35.70523211131943242, -276.9450112145505045, -260.6218447678022017 ) ) ;
#71437=CARTESIAN_POINT ( 'NONE',  ( -4.847791930983072817, -292.6422410391843414, -337.5763733692938899 ) ) ;
#71438=CARTESIAN_POINT ( 'NONE',  ( -87.15567503646454384, -297.5178172236590513, -325.1017967811174003 ) ) ;
#71439=CARTESIAN_POINT ( 'NONE',  ( 31.62965106325087206, -274.6814783460080776, -295.6101805169362251 ) ) ;
#71442=CARTESIAN_POINT ( 'NONE',  ( -114.3167787017339663, -296.2284117409971032, -269.5985106030441329 ) ) ;
#71443=CARTESIAN_POINT ( 'NONE',  ( 34.47759765648295627, -289.7281851577434395, -290.1307548240131950 ) ) ;
#71444=CARTESIAN_POINT ( 'NONE',  ( -60.24766513392076206, -295.7551677297219612, -198.8907321425861312 ) ) ;
#71445=CARTESIAN_POINT ( 'NONE',  ( -5.740868647919679546, -289.2766615644503077, -336.2798567322572580 ) ) ;
#71447=CARTESIAN_POINT ( 'NONE',  ( -90.88543552336295761, -278.3737213555781977, -215.2789469846213990 ) ) ;
#71448=CARTESIAN_POINT ( 'NONE',  ( -3.266480344012961723, -295.2654424718415385, -339.3118489323050539 ) ) ;
#71449=CARTESIAN_POINT ( 'NONE',  ( -90.74498107853588635, -287.9387880582918342, -324.1787346852301539 ) ) ;
#71450=CARTESIAN_POINT ( 'NONE',  ( -79.46184656144620817, -295.9376861448615159, -334.7943202613432163 ) ) ;
#71452=CARTESIAN_POINT ( 'NONE',  ( 31.56141735094734813, -294.2087905507810888, -294.6879012307194330 ) ) ;
#71457=CARTESIAN_POINT ( 'NONE',  ( -3.352018646887067632, -290.1317181207722911, -338.6940567775878321 ) ) ;
#71458=CARTESIAN_POINT ( 'NONE',  ( -37.37352853689063181, -282.5519495502701375, -190.3611179825600175 ) ) ;
#71462=CARTESIAN_POINT ( 'NONE',  ( -31.07378316378691352, -279.4778324171464305, -193.6663023847335126 ) ) ;
#71463=CARTESIAN_POINT ( 'NONE',  ( -36.13915126887679463, -285.0371959840802560, -345.1847927563771350 ) ) ;
#71465=CARTESIAN_POINT ( 'NONE',  ( 30.90374222105522506, -285.6812455088237925, -235.9930239145242012 ) ) ;
#71467=CARTESIAN_POINT ( 'NONE',  ( -48.29659045905209780, -287.2723401326873045, -344.0426568705645991 ) ) ;
#71468=CARTESIAN_POINT ( 'NONE',  ( -5.777417045875322010, -278.5019492286043032, -339.2378304280849761 ) ) ;
#71470=CARTESIAN_POINT ( 'NONE',  ( -109.9661095660103030, -278.6561037714956228, -262.4810183594653950 ) ) ;
#71471=CARTESIAN_POINT ( 'NONE',  ( -96.48329329864841952, -278.5012371238213973, -227.3941001007837031 ) ) ;
#71472=CARTESIAN_POINT ( 'NONE',  ( 35.43225300282824719, -276.3241071104941398, -245.9978551397829563 ) ) ;
#71473=CARTESIAN_POINT ( 'NONE',  ( -96.50093552310204359, -278.0043876351865038, -221.6766356938893523 ) ) ;
#71474=CARTESIAN_POINT ( 'NONE',  ( 23.85752577023820820, -22.80717641334416257, -342.6356047177218329 ) ) ;
#71475=CARTESIAN_POINT ( 'NONE',  ( -27.03999952409519025, -275.1211835814887081, -194.2375214088650068 ) ) ;
#71476=CARTESIAN_POINT ( 'NONE',  ( -82.63601058452800885, -298.8723409525148895, -208.7565020164376506 ) ) ;
#71477=CARTESIAN_POINT ( 'NONE',  ( 21.27581636871892101, -283.4090924074130839, -223.5744983911110353 ) ) ;
#71478=CARTESIAN_POINT ( 'NONE',  ( 82.66537480607564703, -298.2604009065653372, -193.2156244055160528 ) ) ;
#71479=CARTESIAN_POINT ( 'NONE',  ( -9.388194383048595881, -287.5059696358736119, -202.5771506798083124 ) ) ;
#71480=CARTESIAN_POINT ( 'NONE',  ( -0.2309437621850514710, -288.2987939397200989, -204.0381579992571517 ) ) ;
#71481=CARTESIAN_POINT ( 'NONE',  ( 24.31988302674011493, -287.4428948066425278, -309.6261384327821133 ) ) ;
#71482=CARTESIAN_POINT ( 'NONE',  ( -69.16672939997172875, -282.9673061595082117, -340.4233221233238282 ) ) ;
#71483=CARTESIAN_POINT ( 'NONE',  ( 5.402910941885852303, -279.0414961008050909, -210.2001785130106271 ) ) ;
#71484=CARTESIAN_POINT ( 'NONE',  ( -63.01186688303901917, -287.5748632987310316, -200.6506517138367087 ) ) ;
#71485=CARTESIAN_POINT ( 'NONE',  ( 35.01869465258602787, -279.8488280918078317, -256.3417356413095831 ) ) ;
#71486=CARTESIAN_POINT ( 'NONE',  ( -56.71414489996688246, -278.6222334833291825, -341.3079147806263904 ) ) ;
#71488=CARTESIAN_POINT ( 'NONE',  ( 32.15865163379631753, -276.3431858935818468, -292.8930851989941289 ) ) ;
#71489=CARTESIAN_POINT ( 'NONE',  ( -62.64703933424094373, -288.1690947169889796, -342.7196952740434881 ) ) ;
#71490=CARTESIAN_POINT ( 'NONE',  ( -31.63805241721790651, -283.7847380058757381, -347.0009019828759165 ) ) ;
#71491=CARTESIAN_POINT ( 'NONE',  ( -112.9389728075479411, -285.2269463557754534, -255.7806732370833629 ) ) ;
#71492=CARTESIAN_POINT ( 'NONE',  ( 22.11225966026825063, -281.1271147412086293, -228.0028051030079439 ) ) ;
#71496=CARTESIAN_POINT ( 'NONE',  ( 7.227348878636523644, -290.3128700102743096, -331.6949505549666242 ) ) ;
#71497=CARTESIAN_POINT ( 'NONE',  ( -102.7852670100547243, -289.7587127178177298, -230.6302618005856289 ) ) ;
#71498=CARTESIAN_POINT ( 'NONE',  ( -91.28777028412206107, -272.3196671839227179, -220.8124662025029750 ) ) ;
#71499=CARTESIAN_POINT ( 'NONE',  ( 36.19193832824478108, -292.6178860356962446, -247.8640781329650622 ) ) ;
#71500=CARTESIAN_POINT ( 'NONE',  ( -98.69857132884716577, -288.4705046532625374, -311.2012787157181606 ) ) ;
#71501=CARTESIAN_POINT ( 'NONE',  ( 25.72289322775306175, -291.2641713841838396, -231.5232156683388496 ) ) ;
#71502=CARTESIAN_POINT ( 'NONE',  ( 25.28156110685261027, -288.2326344144817654, -232.0798215491795702 ) ) ;
#71503=CARTESIAN_POINT ( 'NONE',  ( -110.4683760289727132, -299.2662352645559167, -253.7030783399848985 ) ) ;
#71504=CARTESIAN_POINT ( 'NONE',  ( -7.686658965846624447, -290.6636682903838391, -339.2631550685158004 ) ) ;
#71505=CARTESIAN_POINT ( 'NONE',  ( -41.91631914476990062, -289.9944572527207924, -195.3337810406539745 ) ) ;
#71506=CARTESIAN_POINT ( 'NONE',  ( -61.74178741097976797, -293.7353735401338781, -199.3869965513158888 ) ) ;
#71507=CARTESIAN_POINT ( 'NONE',  ( -106.7591720747768562, -285.8042952867276654, -246.8650875239355287 ) ) ;
#71508=CARTESIAN_POINT ( 'NONE',  ( 9.945200732662325294, -294.7015614782469584, -211.8649197382757450 ) ) ;
#71511=CARTESIAN_POINT ( 'NONE',  ( 29.18144493974218534, -300.7989061242936941, -194.7795398347321054 ) ) ;
#71512=CARTESIAN_POINT ( 'NONE',  ( -10.92698970840942252, -281.8960514269948590, -338.6413830139247239 ) ) ;
#71513=CARTESIAN_POINT ( 'NONE',  ( 2.132885978195367294, -280.5238692337476323, -334.1928853213923958 ) ) ;
#71514=CARTESIAN_POINT ( 'NONE',  ( -74.53717673322763915, -294.7307916537503729, -337.6565279610424568 ) ) ;
#71515=CARTESIAN_POINT ( 'NONE',  ( 35.62843806190176821, -273.6299134049132249, -257.9029404304777700 ) ) ;
#71516=CARTESIAN_POINT ( 'NONE',  ( -110.4622936750242133, -276.4506186313086005, -284.3818257799994740 ) ) ;
#71517=CARTESIAN_POINT ( 'NONE',  ( -110.7332702738969061, -297.8167188634415652, -274.2238771431095188 ) ) ;
#71518=CARTESIAN_POINT ( 'NONE',  ( 28.00810587870184776, -273.6048782726140871, -230.6618338102382495 ) ) ;
#71519=CARTESIAN_POINT ( 'NONE',  ( -61.18707176432186401, -296.7930531231925784, -340.0338901139157315 ) ) ;
#71521=CARTESIAN_POINT ( 'NONE',  ( -107.6173160520399676, -297.6234925251642949, -250.0156139653211369 ) ) ;
#71522=DIRECTION ( 'NONE',  ( 0.000000000000000000, 0.000000000000000000, -1.000000000000000000 ) ) ;
#71524=CARTESIAN_POINT ( 'NONE',  ( -1.724244142619061115, -284.5418719285844986, -203.9547656202849168 ) ) ;
#71525=CARTESIAN_POINT ( 'NONE',  ( -92.91240329542510779, -273.0589856134864704, -223.0037098112670719 ) ) ;
#71527=CARTESIAN_POINT ( 'NONE',  ( -52.17328396290285752, -285.8674519637603453, -194.7486434589253292 ) ) ;
#71528=CARTESIAN_POINT ( 'NONE',  ( 38.53674002151437605, -287.0556566207039850, -257.3140983458358733 ) ) ;
#71529=CARTESIAN_POINT ( 'NONE',  ( -111.5789622549427378, -298.3630191131977085, -283.5873883096529084 ) ) ;
#71530=CARTESIAN_POINT ( 'NONE',  ( 27.84374650239059079, -291.0600120212583874, -233.5008489501639701 ) ) ;
#71532=CARTESIAN_POINT ( 'NONE',  ( -95.77633964652434884, -278.4239383879316279, -220.4455044279671938 ) ) ;
#71533=CARTESIAN_POINT ( 'NONE',  ( 35.78497577281001440, -290.8380690714490129, -253.7030783399848985 ) ) ;
#71536=CARTESIAN_POINT ( 'NONE',  ( -9.327709826978388463, -285.2215914868312439, -202.5069363119493460 ) ) ;
#71538=CARTESIAN_POINT ( 'NONE',  ( -70.88934232706381522, -287.4945361432881441, -337.4540922527011730 ) ) ;
#71539=CARTESIAN_POINT ( 'NONE',  ( -73.25380238804000044, -299.1675905631590808, -205.8881676291425435 ) ) ;
#71540=CARTESIAN_POINT ( 'NONE',  ( -73.50293477378076545, -281.0072955818818627, -203.0337893677006491 ) ) ;
#71541=CARTESIAN_POINT ( 'NONE',  ( -102.4164048850196451, -295.0786669671501272, -232.2624267701394558 ) ) ;
#71542=CARTESIAN_POINT ( 'NONE',  ( 25.55902995322113824, -282.0622058932659115, -307.5082476223877848 ) ) ;
#71543=CARTESIAN_POINT ( 'NONE',  ( -96.51005562779111813, -296.0558366839032942, -319.6574316830411249 ) ) ;
#71544=CARTESIAN_POINT ( 'NONE',  ( -50.09273146737339033, -299.4066023248960278, -197.7793093073375132 ) ) ;
#71545=CARTESIAN_POINT ( 'NONE',  ( 26.14445379624881483, -283.0143621068036168, -230.3325390352854072 ) ) ;
#71546=CARTESIAN_POINT ( 'NONE',  ( -77.63145088307130948, -296.5557275530918560, -209.1434650964831690 ) ) ;
#71548=CARTESIAN_POINT ( 'NONE',  ( -74.59631179145532087, -285.5299055823111871, -335.1033982902816319 ) ) ;
#71550=CARTESIAN_POINT ( 'NONE',  ( 10.64812456238590777, -290.1952119285920162, -210.2361428286349110 ) ) ;
#71551=CARTESIAN_POINT ( 'NONE',  ( 36.43371240826417079, -274.4772896611304418, -248.6960973273557727 ) ) ;
#71552=CARTESIAN_POINT ( 'NONE',  ( 28.73942239600594917, -292.9650167402072611, -239.2210865081845270 ) ) ;
#71554=CARTESIAN_POINT ( 'NONE',  ( 34.43129487909363462, -282.8538656425229760, -253.6475025022920136 ) ) ;
#71555=CARTESIAN_POINT ( 'NONE',  ( 36.38501525290016048, -277.0963258548464978, -266.0723892975736362 ) ) ;
#71557=CARTESIAN_POINT ( 'NONE',  ( -112.5536940831012060, -285.8038529190048962, -284.1331751001197290 ) ) ;
#71558=CARTESIAN_POINT ( 'NONE',  ( 19.15150624436531857, -279.6859568984608018, -223.4838627648655347 ) ) ;
#71559=CARTESIAN_POINT ( 'NONE',  ( -88.44004290149497649, -279.7686299967593868, -325.2606627201456035 ) ) ;
#71560=CARTESIAN_POINT ( 'NONE',  ( -40.44025748586465596, -298.0143435127642420, -193.3713612973597264 ) ) ;
#71561=CARTESIAN_POINT ( 'NONE',  ( 18.90176012560037222, -276.1027469310284346, -322.9507860096531999 ) ) ;
#71562=CARTESIAN_POINT ( 'NONE',  ( 19.95686336691050400, -296.1332113089037534, -317.8815222580238924 ) ) ;
#71565=CARTESIAN_POINT ( 'NONE',  ( -96.45877731531432175, -294.0463051459646522, -317.7681185191204349 ) ) ;
#71566=CARTESIAN_POINT ( 'NONE',  ( -67.07681387855500077, -273.1591948399645844, -203.6105318771257373 ) ) ;
#71567=CARTESIAN_POINT ( 'NONE',  ( -19.43106419327913770, -296.3460742766268936, -344.5904198241545942 ) ) ;
#71568=CARTESIAN_POINT ( 'NONE',  ( 24.57444020611981017, -295.3591906175447548, -315.4875457036288822 ) ) ;
#71570=CARTESIAN_POINT ( 'NONE',  ( -45.53858600060075190, -291.1564417866723034, -344.7441771258927474 ) ) ;
#71571=CARTESIAN_POINT ( 'NONE',  ( -48.91591296558655699, -275.1996230803521257, -344.3466481428027350 ) ) ;
#71572=CARTESIAN_POINT ( 'NONE',  ( -100.3818052584677218, -279.9350375895110119, -310.0459813418519275 ) ) ;
#71573=CARTESIAN_POINT ( 'NONE',  ( -107.3496476419772279, -294.2996964159375466, -295.8150277207770387 ) ) ;
#71574=CARTESIAN_POINT ( 'NONE',  ( 23.58412914423543683, -282.8042388404967369, -225.3239243514343002 ) ) ;
#71575=CARTESIAN_POINT ( 'NONE',  ( -67.66305006227771912, -284.5649735396472693, -203.6165166077861670 ) ) ;
#71576=CARTESIAN_POINT ( 'NONE',  ( 66.80823473016013736, 46.34870276661032307, -317.8007354683743415 ) ) ;
#71578=CARTESIAN_POINT ( 'NONE',  ( -108.4468605238712087, -283.9990651714399519, -287.0333342115465030 ) ) ;
#71579=CARTESIAN_POINT ( 'NONE',  ( 12.77972700939818651, -281.8122921188626719, -212.3151443872760638 ) ) ;
#71580=CARTESIAN_POINT ( 'NONE',  ( -113.0924092642269727, -283.4947163427395367, -258.6171165374078669 ) ) ;
#71581=CARTESIAN_POINT ( 'NONE',  ( -113.8435366932767465, -279.4060835758023131, -277.3217065339483725 ) ) ;
#71582=CARTESIAN_POINT ( 'NONE',  ( -51.16782384255493099, -278.7459310332778841, -345.4047456536860636 ) ) ;
#71583=CARTESIAN_POINT ( 'NONE',  ( 17.40634833298267736, -296.6948066931273047, -313.9805196606274080 ) ) ;
#71584=CARTESIAN_POINT ( 'NONE',  ( -111.5685550221716511, -271.9231168036148460, -296.3965291073083108 ) ) ;
#71585=ORIENTED_EDGE ( 'NONE', *, *, #33448, .T. ) ;
#71587=CARTESIAN_POINT ( 'NONE',  ( -70.15493457438154223, -299.6199537748950092, -202.9200896783225403 ) ) ;
#71588=CARTESIAN_POINT ( 'NONE',  ( -90.63052692306658287, -277.3129362275749941, -218.0179421694803352 ) ) ;
#71589=CARTESIAN_POINT ( 'NONE',  ( -113.3557315856648557, -292.3371030186479516, -268.4034833780483496 ) ) ;
#71590=CARTESIAN_POINT ( 'NONE',  ( 33.40894805935678136, -292.6582720755254172, -251.9698578426984739 ) ) ;
#71591=CARTESIAN_POINT ( 'NONE',  ( -113.0738433005874413, -289.8890167207642889, -284.0064690308841477 ) ) ;
#71593=CARTESIAN_POINT ( 'NONE',  ( 36.52228909893809572, -292.3736914102457263, -289.9242820855620266 ) ) ;
#71594=CARTESIAN_POINT ( 'NONE',  ( -62.82014232609035531, -284.1148769530660161, -201.0441579418894946 ) ) ;
#71595=CARTESIAN_POINT ( 'NONE',  ( -1.869711445374419467, -294.3876342644962278, -205.1346956712587541 ) ) ;
#71596=CARTESIAN_POINT ( 'NONE',  ( -33.18032793264231373, -284.5852370881650018, -196.7350771420746298 ) ) ;
#71597=CARTESIAN_POINT ( 'NONE',  ( -18.59377739586923894, -284.1209001642205862, -341.4755350446364446 ) ) ;
#71598=EDGE_LOOP ( 'NONE', ( #84491, #7730, #39263, #82832 ) ) ;
#71599=CARTESIAN_POINT ( 'NONE',  ( -56.14279642456811814, -292.7570883067071463, -195.8795997177077481 ) ) ;
#71601=CARTESIAN_POINT ( 'NONE',  ( -38.36100793374497187, -280.5313865153265169, -197.2942786715137800 ) ) ;
#71602=CARTESIAN_POINT ( 'NONE',  ( -11.20717829123565501, -293.5140747523427081, -342.4243038314843943 ) ) ;
#71603=CARTESIAN_POINT ( 'NONE',  ( -8.284700953983888283, -289.4840776078157205, -341.5079751470012184 ) ) ;
#71604=CARTESIAN_POINT ( 'NONE',  ( -96.33982805634261126, -290.3791504547903628, -319.7652302058426130 ) ) ;
#71605=CARTESIAN_POINT ( 'NONE',  ( 15.02801775151314168, -286.9835232321754006, -219.5043322631170781 ) ) ;
#71608=CARTESIAN_POINT ( 'NONE',  ( -34.87080899689524216, -296.8818312747065420, -346.0856198296137904 ) ) ;
#71609=AXIS2_PLACEMENT_3D ( 'NONE', #91391, #11397, #91858 ) ;
#71610=CARTESIAN_POINT ( 'NONE',  ( -108.4241622780869676, -295.5998369217901995, -241.9242758961994184 ) ) ;
#71611=CARTESIAN_POINT ( 'NONE',  ( -109.8530493278866800, -277.7505861745600555, -259.7377054285277040 ) ) ;
#71612=CARTESIAN_POINT ( 'NONE',  ( -46.86716050204879735, -273.4419225846557993, -194.0145888683066175 ) ) ;
#71613=CARTESIAN_POINT ( 'NONE',  ( -72.47198465341396911, -294.0058772578710204, -335.1564694544476311 ) ) ;
#71614=CARTESIAN_POINT ( 'NONE',  ( 10.11792469851334708, -276.4766671076706075, -213.5000237227767741 ) ) ;
#71615=CARTESIAN_POINT ( 'NONE',  ( -97.26463535932182936, -271.2961678713374454, -226.4567184861905673 ) ) ;
#71616=CARTESIAN_POINT ( 'NONE',  ( 33.68862166955093329, -294.5144608013111451, -251.8726380246564815 ) ) ;
#71617=CARTESIAN_POINT ( 'NONE',  ( -96.65043022234222292, -297.0310624997503623, -313.4719879698985210 ) ) ;
#71620=CARTESIAN_POINT ( 'NONE',  ( -110.4843634630860549, -294.7739764931605464, -253.0354367145798449 ) ) ;
#71621=CARTESIAN_POINT ( 'NONE',  ( -37.61563500620392375, -298.7002158081417633, -193.4635383920897880 ) ) ;
#71622=CARTESIAN_POINT ( 'NONE',  ( -70.25215340441238254, -288.0693311842300091, -336.1951258724580498 ) ) ;
#71623=CARTESIAN_POINT ( 'NONE',  ( -112.3417001281295029, -274.5519907608264134, -270.3865269787834222 ) ) ;
#71624=CARTESIAN_POINT ( 'NONE',  ( -67.51728771384556183, -274.1591084404207095, -199.5871056813758457 ) ) ;
#71625=CARTESIAN_POINT ( 'NONE',  ( -103.9541643660616757, -296.4811144576833044, -300.3990324955398137 ) ) ;
#71626=CARTESIAN_POINT ( 'NONE',  ( -107.0019747050131826, -280.9052485870719238, -241.6234606999778407 ) ) ;
#71627=CARTESIAN_POINT ( 'NONE',  ( 35.13647504956216494, -280.5494270097165668, -295.0248807746287412 ) ) ;
#71629=CARTESIAN_POINT ( 'NONE',  ( -81.50980137050387953, -282.9840380006575060, -333.3742277718313858 ) ) ;
#71630=CARTESIAN_POINT ( 'NONE',  ( 38.62820432524579672, -274.7505092193504765, -258.3645751439145783 ) ) ;
#71631=CARTESIAN_POINT ( 'NONE',  ( -5.262046132045552049, -278.8671928222951237, -201.2428409666093216 ) ) ;
#71632=CARTESIAN_POINT ( 'NONE',  ( -17.45199622606810763, -278.3080528031024983, -197.8736838824151789 ) ) ;
#71633=CARTESIAN_POINT ( 'NONE',  ( -105.9591363085006464, -271.4810009299662283, -243.6307527733444829 ) ) ;
#71634=CARTESIAN_POINT ( 'NONE',  ( 33.41221441907261180, -277.2283432157170182, -245.3296959945814990 ) ) ;
#71636=CARTESIAN_POINT ( 'NONE',  ( 28.06086145274387178, -291.0753804406915606, -232.9323624706967450 ) ) ;
#71637=CARTESIAN_POINT ( 'NONE',  ( -58.93868409273427744, -291.7802225772009024, -196.4519150127638341 ) ) ;
#71638=CARTESIAN_POINT ( 'NONE',  ( 15.68050772243511481, -278.3045312274953744, -323.7130314501222301 ) ) ;
#71639=CARTESIAN_POINT ( 'NONE',  ( 0.4838307566632938372, -272.5559825923679682, -205.5832506019904997 ) ) ;
#71641=CARTESIAN_POINT ( 'NONE',  ( -92.72255597985856923, -283.2586749062211311, -219.7101000446822070 ) ) ;
#71643=CARTESIAN_POINT ( 'NONE',  ( 19.99438012179129487, -292.9910809704343819, -316.2036794160327986 ) ) ;
#71644=CARTESIAN_POINT ( 'NONE',  ( 35.97547383269628085, -285.8437597006701480, -282.0805864867554078 ) ) ;
#71647=CARTESIAN_POINT ( 'NONE',  ( -85.78893436411632933, -293.7223037626031896, -327.6819781360918569 ) ) ;
#71648=CARTESIAN_POINT ( 'NONE',  ( -83.47952874564877845, -282.1513635884786595, -331.2058617852938482 ) ) ;
#71649=CARTESIAN_POINT ( 'NONE',  ( -107.9988771690913865, -280.4313223872106846, -249.0537542717651149 ) ) ;
#71650=CARTESIAN_POINT ( 'NONE',  ( -113.2039295395671559, -285.6189284043271073, -281.3621415188760011 ) ) ;
#71651=CARTESIAN_POINT ( 'NONE',  ( -17.23822585400530727, -278.5480334327500600, -197.0820327427349241 ) ) ;
#71652=CARTESIAN_POINT ( 'NONE',  ( 11.13405799563638432, -286.7454904218800493, -215.7120609333748575 ) ) ;
#71654=CARTESIAN_POINT ( 'NONE',  ( -32.36270670230294400, -278.4135632189978651, -343.8320874678398127 ) ) ;
#71655=CARTESIAN_POINT ( 'NONE',  ( -108.1314139690347105, -279.5989871059999246, -251.8343779645686595 ) ) ;
#71656=CARTESIAN_POINT ( 'NONE',  ( -103.9893939049711946, -286.9972294998182747, -235.0855380251324789 ) ) ;
#71659=CARTESIAN_POINT ( 'NONE',  ( -80.62326767628746893, -297.3164989121188455, -206.6125872719093763 ) ) ;
#71660=CARTESIAN_POINT ( 'NONE',  ( -5.058756500323404737, -290.6049254231585905, -337.6638546134918215 ) ) ;
#71662=CARTESIAN_POINT ( 'NONE',  ( -115.3430155898818299, -281.2662352645559167, -252.5904736702033517 ) ) ;
#71664=CARTESIAN_POINT ( 'NONE',  ( -64.22014028701661914, -271.7021451115908235, -200.1505636657080913 ) ) ;
#71665=CARTESIAN_POINT ( 'NONE',  ( 14.90463326366642782, -291.1734704565086531, -214.8200912840153478 ) ) ;
#71666=CARTESIAN_POINT ( 'NONE',  ( -69.75700534964708766, -294.9986136034382866, -335.8381095846580706 ) ) ;
#71668=CARTESIAN_POINT ( 'NONE',  ( 32.49149305582440661, -288.7625260792373751, -246.8232148925967806 ) ) ;
#71669=CARTESIAN_POINT ( 'NONE',  ( 20.45344296845333076, -282.6679971410620738, -224.1258992502960155 ) ) ;
#71670=CARTESIAN_POINT ( 'NONE',  ( -109.3044470916250646, -291.6488725461564968, -296.2077444525777423 ) ) ;
#71671=CARTESIAN_POINT ( 'NONE',  ( -107.2737544383766419, -291.4673105193938341, -301.5204688082704365 ) ) ;
#71672=CARTESIAN_POINT ( 'NONE',  ( -110.0253345029112779, -286.3146966461031866, -288.8567916984801514 ) ) ;
#71673=CARTESIAN_POINT ( 'NONE',  ( -96.14781653577701093, -278.0489294418554778, -320.0890195875368818 ) ) ;
#71674=CARTESIAN_POINT ( 'NONE',  ( 24.52136526099614144, -292.2169197850424780, -313.7688859149677683 ) ) ;
#71675=CARTESIAN_POINT ( 'NONE',  ( 29.28764477213070094, -280.8835762765841082, -231.7666831161311052 ) ) ;
#71676=AXIS2_PLACEMENT_3D ( 'NONE', #59649, #59165, #32140 ) ;
#71677=CARTESIAN_POINT ( 'NONE',  ( -93.86949603807366316, -275.0857538483523399, -222.2221177736223297 ) ) ;
#71680=CARTESIAN_POINT ( 'NONE',  ( 21.27581636871892101, -295.4090924074130839, -223.5744983911110353 ) ) ;
#71681=CARTESIAN_POINT ( 'NONE',  ( 23.67967844883697026, -273.1819578725408633, -225.0801576086992384 ) ) ;
#71683=CARTESIAN_POINT ( 'NONE',  ( -4.314145064791616413, -280.0073286965790089, -205.1769067137720697 ) ) ;
#71685=CARTESIAN_POINT ( 'NONE',  ( 24.05863392048273397, -277.3696781411160828, -316.1651319809926690 ) ) ;
#71686=CARTESIAN_POINT ( 'NONE',  ( -98.95074209796707976, -298.5317832405259537, -230.0233642950922217 ) ) ;
#71687=CARTESIAN_POINT ( 'NONE',  ( -47.23793639681001366, -282.2337233190768870, -346.4852581763551029 ) ) ;
#71688=CARTESIAN_POINT ( 'NONE',  ( -110.4160519150708240, -292.1583542538229494, -282.1928394263150039 ) ) ;
#71689=CARTESIAN_POINT ( 'NONE',  ( -91.61372663536592142, -274.8946426137387107, -216.8729178494533585 ) ) ;
#71690=CARTESIAN_POINT ( 'NONE',  ( -55.23463433823114599, -275.1418104653753858, -195.9760309235535090 ) ) ;
#71692=CARTESIAN_POINT ( 'NONE',  ( 9.392485132521358082, -296.4087377666173211, -328.8738142022788224 ) ) ;
#71693=CARTESIAN_POINT ( 'NONE',  ( -71.06332043049040692, -281.4980089476669036, -337.1802455307663990 ) ) ;
#71694=CARTESIAN_POINT ( 'NONE',  ( -113.3398548395350076, -290.0656463711811739, -282.6095779671533137 ) ) ;
#71695=CARTESIAN_POINT ( 'NONE',  ( 35.17864991614144543, -273.8010451705940227, -288.0966731952875648 ) ) ;
#71696=CARTESIAN_POINT ( 'NONE',  ( 13.69578042214607549, -288.3530144382849016, -213.7075207084152453 ) ) ;
#71698=CARTESIAN_POINT ( 'NONE',  ( -109.0098733389127403, -289.6750882933995968, -254.9371423846353935 ) ) ;
#71700=CARTESIAN_POINT ( 'NONE',  ( -96.99211262239884945, -289.7715144920263697, -222.6072219637948422 ) ) ;
#71701=CARTESIAN_POINT ( 'NONE',  ( -107.0205207128411189, -290.5087291010706849, -248.4798317883383163 ) ) ;
#71703=CARTESIAN_POINT ( 'NONE',  ( 38.66707351460367903, -288.5036681321446395, -260.1552942077444754 ) ) ;
#71704=CARTESIAN_POINT ( 'NONE',  ( 20.85634145735024347, -276.5050219194279180, -314.4641274317513648 ) ) ;
#71706=CARTESIAN_POINT ( 'NONE',  ( -24.97127819426458828, -293.8183886548726491, -346.1015899336565553 ) ) ;
#71707=CARTESIAN_POINT ( 'NONE',  ( -55.66983819907394349, -283.9335075615382493, -345.0430578416849130 ) ) ;
#71708=CARTESIAN_POINT ( 'NONE',  ( -97.56651273162216853, -285.5274993009537070, -222.4161887559072568 ) ) ;
#71709=CARTESIAN_POINT ( 'NONE',  ( -36.18894229743908397, -283.3705864035105151, -343.3731624427013571 ) ) ;
#71710=CARTESIAN_POINT ( 'NONE',  ( 203.5338562182569149, 295.8836489450777094, -54.00000000004095568 ) ) ;
#71711=CARTESIAN_POINT ( 'NONE',  ( 201.9871130242204345, 295.7236060444520263, -68.57413240043143787 ) ) ;
#71712=CARTESIAN_POINT ( 'NONE',  ( 152.0738250329050345, 205.6678486289000602, -214.6699954404999175 ) ) ;
#71713=CARTESIAN_POINT ( 'NONE',  ( -11.42347044757535102, -273.5956507169744327, -201.8902325781756986 ) ) ;
#71714=CARTESIAN_POINT ( 'NONE',  ( 22.54124422908810388, -273.8844686918206435, -228.0515702116383068 ) ) ;
#71715=CARTESIAN_POINT ( 'NONE',  ( -109.3821301432877817, -295.7161436859888681, -297.5244840198336647 ) ) ;
#71716=CARTESIAN_POINT ( 'NONE',  ( 203.1406098482175082, 291.9636561924038460, -68.25767031306274646 ) ) ;
#71717=CARTESIAN_POINT ( 'NONE',  ( -64.70794031982967454, -272.3870210641824769, -198.9020305056669145 ) ) ;
#71718=CARTESIAN_POINT ( 'NONE',  ( -104.8515973134611556, -298.8234751508008458, -239.3620821199822046 ) ) ;
#71719=CARTESIAN_POINT ( 'NONE',  ( 29.88288232784202592, -289.2658341984018762, -300.1875965994962030 ) ) ;
#71720=CARTESIAN_POINT ( 'NONE',  ( -75.15076886893835706, -292.6155511243106275, -207.4949966826860930 ) ) ;
#71722=CARTESIAN_POINT ( 'NONE',  ( -105.0517392887751527, -297.9634991113347837, -234.0796786594165155 ) ) ;
#71723=CARTESIAN_POINT ( 'NONE',  ( -12.00651713241685670, -286.8833571480352020, -201.8328979252069928 ) ) ;
#71724=CARTESIAN_POINT ( 'NONE',  ( 39.34175060679670111, -294.4258670534229623, -276.0170551198291378 ) ) ;
#71725=CARTESIAN_POINT ( 'NONE',  ( -86.35129232163889412, -296.2041091161521535, -329.6703649519598116 ) ) ;
#71726=CARTESIAN_POINT ( 'NONE',  ( 33.30766822546267747, -293.4762330291529793, -251.9854069548942448 ) ) ;
#71727=VERTEX_POINT ( 'NONE', #78946 ) ;
#71728=CARTESIAN_POINT ( 'NONE',  ( -31.39818384300815168, -276.0467811391014834, -195.0222009776275911 ) ) ;
#71730=CARTESIAN_POINT ( 'NONE',  ( -73.73099912836624981, -279.0899859423332714, -202.5571996825050860 ) ) ;
#71731=CARTESIAN_POINT ( 'NONE',  ( 22.94600557011623110, -273.3640957574764911, -227.7736029834128999 ) ) ;
#71732=CARTESIAN_POINT ( 'NONE',  ( -68.42610636966820437, -274.7136067350936059, -203.9546977671403170 ) ) ;
#71734=CARTESIAN_POINT ( 'NONE',  ( 35.83769547813096779, -276.5453796724441986, -274.3134172970944746 ) ) ;
#71735=CARTESIAN_POINT ( 'NONE',  ( 36.29758806142450567, -277.0746468417739266, -251.6200067206809763 ) ) ;
#71736=CARTESIAN_POINT ( 'NONE',  ( 38.06127762496454636, -273.5827152938435347, -271.1794932906690860 ) ) ;
#71737=CARTESIAN_POINT ( 'NONE',  ( -110.2000743452557572, -297.1172064540436963, -276.9170275267924239 ) ) ;
#71738=CARTESIAN_POINT ( 'NONE',  ( -26.13544043930307126, -293.4814049398514157, -343.0920925375120873 ) ) ;
#71740=CARTESIAN_POINT ( 'NONE',  ( -77.46577931404308970, -280.0217816100312689, -204.6520080396967671 ) ) ;
#71741=CARTESIAN_POINT ( 'NONE',  ( 32.09883516742757337, -276.0175712705664068, -292.8780463338557638 ) ) ;
#71742=TOROIDAL_SURFACE ( 'NONE', #30888, 5.343514653206205445, 1.000000000000000000 ) ;
#71743=CARTESIAN_POINT ( 'NONE',  ( -1.187718770075380625, -285.2064826773611230, -202.9356932109756713 ) ) ;
#71744=CARTESIAN_POINT ( 'NONE',  ( -37.28125707365905583, -300.0530651684923669, -195.1936765916527463 ) ) ;
#71745=CARTESIAN_POINT ( 'NONE',  ( 82.62898823957701211, -301.1181951566114208, -197.3182997069781948 ) ) ;
#71746=AXIS2_PLACEMENT_3D ( 'NONE', #56748, #21669, #35876 ) ;
#71747=CARTESIAN_POINT ( 'NONE',  ( 31.99688712007001001, -286.4399460987569910, -247.0209799082480515 ) ) ;
#71749=CARTESIAN_POINT ( 'NONE',  ( -84.06025536891111472, -277.6401271231392798, -212.8896557090281760 ) ) ;
#71750=CARTESIAN_POINT ( 'NONE',  ( -71.19671980122386401, -278.1708654903962383, -205.0077067614502937 ) ) ;
#71751=CARTESIAN_POINT ( 'NONE',  ( -36.52480683115501847, -285.0420590774318157, -345.3692216833477460 ) ) ;
#71752=CARTESIAN_POINT ( 'NONE',  ( -89.35644591605554865, -279.0094471131884575, -322.2174095497524036 ) ) ;
#71754=AXIS2_PLACEMENT_3D ( 'NONE', #47338, #40694, #92310 ) ;
#71755=CARTESIAN_POINT ( 'NONE',  ( 14.32561868106340519, -274.7405479958995898, -326.4412052992155395 ) ) ;
#71756=CARTESIAN_POINT ( 'NONE',  ( 5.229381813058770589, -275.2962646132127134, -210.8713289407209004 ) ) ;
#71757=CARTESIAN_POINT ( 'NONE',  ( 27.68744924600936130, -283.0500678239332046, -232.6618055744356184 ) ) ;
#71759=CARTESIAN_POINT ( 'NONE',  ( 35.40480076664930209, -289.7337065991507643, -290.8355867802104626 ) ) ;
#71760=CARTESIAN_POINT ( 'NONE',  ( 36.88031470064380102, -291.6914703853266815, -281.2241205064065639 ) ) ;
#71762=CARTESIAN_POINT ( 'NONE',  ( 82.14511625994450128, -299.8483204291535458, -197.3559792037316356 ) ) ;
#71763=CARTESIAN_POINT ( 'NONE',  ( -3.865200399341448101, -273.1881556656844054, -204.9209433488237835 ) ) ;
#71764=CARTESIAN_POINT ( 'NONE',  ( 31.99032694162384161, -291.3432971920728392, -243.8293351380426657 ) ) ;
#71765=CARTESIAN_POINT ( 'NONE',  ( 180.5468918863934960, 256.3577768311903355, -167.2605672291198857 ) ) ;
#71767=CARTESIAN_POINT ( 'NONE',  ( -113.4228607040191719, -288.9498270393111170, -276.8749633338974832 ) ) ;
#71768=CARTESIAN_POINT ( 'NONE',  ( -93.15089247011005114, -285.4714811356282098, -318.6687930223515082 ) ) ;
#71769=CARTESIAN_POINT ( 'NONE',  ( -10.33289605331482086, -284.6395534953461492, -199.2804243918201053 ) ) ;
#71770=CARTESIAN_POINT ( 'NONE',  ( -13.32001105019807419, -284.1593826679187487, -339.9732896615436744 ) ) ;
#71771=CARTESIAN_POINT ( 'NONE',  ( -110.5519284178350432, -285.3476241554911894, -270.9207150378398978 ) ) ;
#71772=CARTESIAN_POINT ( 'NONE',  ( -94.43165724661248817, -293.2108330865286234, -221.1565965264391593 ) ) ;
#71773=CARTESIAN_POINT ( 'NONE',  ( -0.05940419736651295773, -274.8675158897616484, -202.9979689485211907 ) ) ;
#71774=CARTESIAN_POINT ( 'NONE',  ( -105.2306614181790394, -288.1965610808502447, -303.6524513911197687 ) ) ;
#71775=CARTESIAN_POINT ( 'NONE',  ( -93.33399293753780057, -277.8297409066191790, -323.2946352185534238 ) ) ;
#71776=CARTESIAN_POINT ( 'NONE',  ( 25.83246074067539766, -296.0702777093330269, -310.2184456057734110 ) ) ;
#71778=CARTESIAN_POINT ( 'NONE',  ( -106.6379572354042296, -298.6233781216988632, -303.7686719486574702 ) ) ;
#71779=CARTESIAN_POINT ( 'NONE',  ( -89.25441501243226128, -282.4860578409909522, -322.4548065540936932 ) ) ;
#71780=CARTESIAN_POINT ( 'NONE',  ( -38.12284122492987848, -278.0422048612285266, -195.3651816150428147 ) ) ;
#71781=CARTESIAN_POINT ( 'NONE',  ( 18.67717997959611509, -297.1422734259927552, -194.1760574865865578 ) ) ;
#71782=CARTESIAN_POINT ( 'NONE',  ( 16.60077602297621624, -275.6076851503423200, -319.7164042526050594 ) ) ;
#71783=CARTESIAN_POINT ( 'NONE',  ( -36.21476309781461111, -293.5866219212883266, -196.6638040726873271 ) ) ;
#71784=CARTESIAN_POINT ( 'NONE',  ( 32.85116189184988400, -294.2157563226932098, -249.2969822167947314 ) ) ;
#71785=CARTESIAN_POINT ( 'NONE',  ( -90.35819045901187962, -297.0984566409026115, -325.5933545764800101 ) ) ;
#71786=CARTESIAN_POINT ( 'NONE',  ( -84.47972061007992295, -295.5554891598225709, -326.1680224458586963 ) ) ;
#71787=CARTESIAN_POINT ( 'NONE',  ( -12.60483822100766638, -290.7306689651027227, -341.1642839473477125 ) ) ;
#71788=CARTESIAN_POINT ( 'NONE',  ( -94.39772701254746323, -284.0162330430446787, -322.0876337816351906 ) ) ;
#71789=CARTESIAN_POINT ( 'NONE',  ( 20.91651007074587199, -273.0296657700174023, -221.9226371214035964 ) ) ;
#71790=CARTESIAN_POINT ( 'NONE',  ( 39.70243564528419711, -287.4003836784361283, -271.5534072559087804 ) ) ;
#71791=CARTESIAN_POINT ( 'NONE',  ( -39.17341128849477627, -279.0551466767266220, -344.9834446690304617 ) ) ;
#71793=CARTESIAN_POINT ( 'NONE',  ( -6.907823991882188430, -285.5203864706758168, -203.7351273666220948 ) ) ;
#71794=CARTESIAN_POINT ( 'NONE',  ( -5.213529017842083668, -286.6291991916397706, -338.1452803980457134 ) ) ;
#71795=CARTESIAN_POINT ( 'NONE',  ( 6.757860130087521178, -59.91093500391586701, -350.7441993381422094 ) ) ;
#71796=CARTESIAN_POINT ( 'NONE',  ( -39.96985841273527740, -285.5258924766216069, -197.3468644025854815 ) ) ;
#71797=CARTESIAN_POINT ( 'NONE',  ( -58.41062556564010322, -284.2591540747295653, -344.2332485280205105 ) ) ;
#71798=CARTESIAN_POINT ( 'NONE',  ( -77.03729641764570601, -290.5931043268431040, -204.5953297476051773 ) ) ;
#71799=CARTESIAN_POINT ( 'NONE',  ( -56.37671641447296622, -281.4111123504840180, -196.5224822393548152 ) ) ;
#71800=CARTESIAN_POINT ( 'NONE',  ( -102.9970570815455062, -280.3839199487563860, -230.9812036140839666 ) ) ;
#71801=CARTESIAN_POINT ( 'NONE',  ( -11.74115963651981431, -280.2281699228663001, -201.9438366833783789 ) ) ;
#71802=CARTESIAN_POINT ( 'NONE',  ( -66.47790118651256819, -275.6485854813661831, -201.6375514828009159 ) ) ;
#71803=CARTESIAN_POINT ( 'NONE',  ( -33.43483734184238187, -295.0042770022172363, -347.2750593515710307 ) ) ;
#71804=CARTESIAN_POINT ( 'NONE',  ( -37.29166841799597165, -287.0716328945454734, -345.0059055043241187 ) ) ;
#71806=CARTESIAN_POINT ( 'NONE',  ( -94.12886339872447650, -292.8486873343707089, -219.5510943273570774 ) ) ;
#71807=CARTESIAN_POINT ( 'NONE',  ( -88.33090852815483629, -296.2379229793014019, -217.6183804543549059 ) ) ;
#71808=CARTESIAN_POINT ( 'NONE',  ( 19.61157610432797682, -284.1401972384553574, -318.3146023257164074 ) ) ;
#71809=CARTESIAN_POINT ( 'NONE',  ( -95.62377097541222781, -295.6008385683056190, -314.3736224449548331 ) ) ;
#71810=CARTESIAN_POINT ( 'NONE',  ( -19.47219931230847934, -293.3563255569554826, -195.7265381718005415 ) ) ;
#71812=CARTESIAN_POINT ( 'NONE',  ( -6.734302065397562487, -281.1162920441148572, -203.9616130972737267 ) ) ;
#71814=CARTESIAN_POINT ( 'NONE',  ( -3.917687623041965495, -273.5410258234661001, -201.2405341016468867 ) ) ;
#71815=CARTESIAN_POINT ( 'NONE',  ( -78.07536641740080086, -290.2354931316477291, -335.6465472546024671 ) ) ;
#71816=CARTESIAN_POINT ( 'NONE',  ( -103.3526660253210565, -282.2001359180881082, -307.6542321543950607 ) ) ;
#71817=CARTESIAN_POINT ( 'NONE',  ( -113.6457656654463761, -291.0175439808587612, -259.8004684760299483 ) ) ;
#71818=CARTESIAN_POINT ( 'NONE',  ( 22.76971771980765169, -288.4628996621580654, -311.8404260667226708 ) ) ;
#71820=CARTESIAN_POINT ( 'NONE',  ( 178.1189667068858000, 253.6096096343568718, -165.4786255472319851 ) ) ;
#71821=CARTESIAN_POINT ( 'NONE',  ( 160.8675658356268343, 217.7272039891784061, -202.3614854212502507 ) ) ;
#71823=CARTESIAN_POINT ( 'NONE',  ( 21.31550574532286291, -278.4094976428775681, -223.6242672951989618 ) ) ;
#71824=CARTESIAN_POINT ( 'NONE',  ( -109.0434605104278916, -277.9415497043815435, -255.7566106584714305 ) ) ;
#71826=CARTESIAN_POINT ( 'NONE',  ( -94.17147791813980007, -278.1252562387663261, -224.0512655645141251 ) ) ;
#71827=CARTESIAN_POINT ( 'NONE',  ( 26.12953847396074636, -274.6436266326655868, -226.7815111782266229 ) ) ;
#71828=CARTESIAN_POINT ( 'NONE',  ( 200.6534333971687545, 286.0685513885803175, -96.65979452701760977 ) ) ;
#71829=CARTESIAN_POINT ( 'NONE',  ( -88.52321589316306927, -277.9255405016471059, -213.6243685558584389 ) ) ;
#71830=CARTESIAN_POINT ( 'NONE',  ( 10.95412489501575237, -280.4006190535507699, -327.3444478219906841 ) ) ;
#71831=CARTESIAN_POINT ( 'NONE',  ( -102.9858506830102982, -298.8180980861067155, -231.9844126909268596 ) ) ;
#71833=CARTESIAN_POINT ( 'NONE',  ( 20.22751120956337090, -293.4106919018047392, -225.3544864841448430 ) ) ;
#71834=VERTEX_POINT ( 'NONE', #6522 ) ;
#71835=CARTESIAN_POINT ( 'NONE',  ( 16.35993724086789669, -286.9544814030525686, -320.6090373511225380 ) ) ;
#71836=CARTESIAN_POINT ( 'NONE',  ( 37.84397290280745096, -276.0006901711001888, -254.1611371329152576 ) ) ;
#71837=CARTESIAN_POINT ( 'NONE',  ( -109.5827616559154478, -272.6952085234271408, -259.5166644620624652 ) ) ;
#71840=CARTESIAN_POINT ( 'NONE',  ( 23.93337300590344796, -282.0751160316062851, -230.0254482823178250 ) ) ;
#71841=CARTESIAN_POINT ( 'NONE',  ( -42.38547125463780674, -281.7494994651199818, -194.5420281233098763 ) ) ;
#71842=CARTESIAN_POINT ( 'NONE',  ( -109.2127080932688727, -283.4258861820418929, -284.4311806257383068 ) ) ;
#71843=CARTESIAN_POINT ( 'NONE',  ( 36.66240991557043571, -283.4965634792587252, -276.8356852629276545 ) ) ;
#71844=CARTESIAN_POINT ( 'NONE',  ( -8.484855210382525215, -275.1473203404668766, -338.1832693540746391 ) ) ;
#71847=CARTESIAN_POINT ( 'NONE',  ( -9.261289996373720967, -277.4970613775752781, -341.8848859715651543 ) ) ;
#71849=CARTESIAN_POINT ( 'NONE',  ( -95.71092465805593008, -276.4572345150953083, -319.6929802806191105 ) ) ;
#71852=CARTESIAN_POINT ( 'NONE',  ( -94.07932934483878284, -285.8466524513269746, -319.9519259584895963 ) ) ;
#71853=CARTESIAN_POINT ( 'NONE',  ( 34.87498181864536662, -292.5940224921241111, -258.5629605926766317 ) ) ;
#71854=CARTESIAN_POINT ( 'NONE',  ( -9.607842461548836255, -288.0477173232401356, -342.0838195875194856 ) ) ;
#71855=CARTESIAN_POINT ( 'NONE',  ( -11.64949625698807267, -284.6312320025913891, -200.9501341726753481 ) ) ;
#71856=CARTESIAN_POINT ( 'NONE',  ( -84.00762512323545650, -283.9713642507327904, -213.3944268964577304 ) ) ;
#71857=CARTESIAN_POINT ( 'NONE',  ( -69.21438447158695340, -287.7171972962955806, -337.1601150514024425 ) ) ;
#71858=CARTESIAN_POINT ( 'NONE',  ( 34.03990156219499852, -282.9820533688626369, -287.4967131971842491 ) ) ;
#71859=CARTESIAN_POINT ( 'NONE',  ( -49.37264000728440294, -271.8987596729892857, -196.2799532956359769 ) ) ;
#71860=CARTESIAN_POINT ( 'NONE',  ( -111.7483806585477737, -282.7443390403341255, -286.7954208593439489 ) ) ;
#71861=CARTESIAN_POINT ( 'NONE',  ( -94.95819166640239928, -297.8890205352169005, -318.3950405513293163 ) ) ;
#71862=CARTESIAN_POINT ( 'NONE',  ( -88.61657461520258039, -283.3351405280789095, -215.3274922950619725 ) ) ;
#71863=CARTESIAN_POINT ( 'NONE',  ( -95.80680844947880814, -280.1111808145026316, -226.2354279263412877 ) ) ;
#71864=CARTESIAN_POINT ( 'NONE',  ( 33.35702277406612382, -289.8843162584950619, -296.0414864011003147 ) ) ;
#71867=CARTESIAN_POINT ( 'NONE',  ( 37.19001511173541985, -295.6316360208157903, -282.8629346609000095 ) ) ;
#71868=CARTESIAN_POINT ( 'NONE',  ( -94.26065944382695250, -275.8752571861291472, -319.1999623771977781 ) ) ;
#71869=CARTESIAN_POINT ( 'NONE',  ( -109.7169137284815292, -289.4211266837438643, -296.3256483703961521 ) ) ;
#71870=CARTESIAN_POINT ( 'NONE',  ( -53.34246703258771305, -293.6605142541033615, -342.4582160637586981 ) ) ;
#71871=CARTESIAN_POINT ( 'NONE',  ( -83.73617232210561667, -278.0850227333908720, -213.2970478755840986 ) ) ;
#71872=CARTESIAN_POINT ( 'NONE',  ( -44.66779988183058947, -296.0981804581261940, -196.4370623990203057 ) ) ;
#71873=CARTESIAN_POINT ( 'NONE',  ( -14.71034408175546204, -293.6668524809140308, -200.4392673152705697 ) ) ;
#71874=CARTESIAN_POINT ( 'NONE',  ( -20.25526795762937127, -282.7662352645559736, -195.3538533559490702 ) ) ;
#71875=CARTESIAN_POINT ( 'NONE',  ( -55.92037789959892535, -293.7670642906631429, -344.3715259207385770 ) ) ;
#71876=CARTESIAN_POINT ( 'NONE',  ( -45.43010981144384886, -290.7564741773368837, -343.7165407087683775 ) ) ;
#71877=CARTESIAN_POINT ( 'NONE',  ( -66.60422421857569475, -289.9139373957862631, -200.2349552563926238 ) ) ;
#71879=CARTESIAN_POINT ( 'NONE',  ( -64.01769526253177389, -290.8321761863759889, -338.9997427166684361 ) ) ;
#71881=CARTESIAN_POINT ( 'NONE',  ( -21.08353462347372442, -289.6409983149790150, -341.6932550656483727 ) ) ;
#71883=CARTESIAN_POINT ( 'NONE',  ( -87.11472619302482201, -290.9323324330699734, -328.6601051939372269 ) ) ;
#71884=CARTESIAN_POINT ( 'NONE',  ( 34.04266256342511809, -279.8848159900762198, -294.6618718617010018 ) ) ;
#71885=CARTESIAN_POINT ( 'NONE',  ( -108.4274720254899762, -290.7719533778829373, -253.6989850963954893 ) ) ;
#71886=CARTESIAN_POINT ( 'NONE',  ( -88.92042349984600946, -279.6838108229380850, -213.2176180303639228 ) ) ;
#71887=CARTESIAN_POINT ( 'NONE',  ( 28.28475668372531615, -281.7458690025740111, -310.6978371835860457 ) ) ;
#71889=CARTESIAN_POINT ( 'NONE',  ( 23.63203378177306035, -284.9568857978640608, -226.6019693509999797 ) ) ;
#71891=CARTESIAN_POINT ( 'NONE',  ( -4.298279218856092321, -280.7514058464799405, -336.8366609902617483 ) ) ;
#71892=CARTESIAN_POINT ( 'NONE',  ( -109.0071855195683952, -282.8391623291549877, -248.0718385701079001 ) ) ;
#71894=CARTESIAN_POINT ( 'NONE',  ( -99.90821221285212062, -276.4493755390499814, -314.0433720304047824 ) ) ;
#71896=CARTESIAN_POINT ( 'NONE',  ( -102.6620246555613676, -282.9451772856358502, -310.5450415452747848 ) ) ;
#71897=CARTESIAN_POINT ( 'NONE',  ( -81.17591050855962465, -274.2422788104820484, -211.7214055761884879 ) ) ;
#71899=CARTESIAN_POINT ( 'NONE',  ( -97.42440885179496490, -292.7455245028399986, -227.4201435665535200 ) ) ;
#71900=CARTESIAN_POINT ( 'NONE',  ( -13.26548193127009867, -275.7841581728339406, -197.8425547780395277 ) ) ;
#71901=CARTESIAN_POINT ( 'NONE',  ( -3.861551987416893095, -276.2643958327149107, -335.2546243397504213 ) ) ;
#71902=CARTESIAN_POINT ( 'NONE',  ( 17.64225064007190014, -296.2658354164618117, -321.3686253435952267 ) ) ;
#71903=CARTESIAN_POINT ( 'NONE',  ( -73.17198516148800991, -289.6804673459489550, -338.5315099698282211 ) ) ;
#71904=CARTESIAN_POINT ( 'NONE',  ( 36.14210674182381666, -279.8568528140182821, -288.0072607088792438 ) ) ;
#71905=CARTESIAN_POINT ( 'NONE',  ( -53.38724561063450835, -291.6852795057395156, -194.9969898139930820 ) ) ;
#71906=CARTESIAN_POINT ( 'NONE',  ( -90.92318618272561537, -290.3266465976862492, -220.4183092012162319 ) ) ;
#71907=CARTESIAN_POINT ( 'NONE',  ( -66.17960405431155380, -293.4294178791556078, -339.6091639940609639 ) ) ;
#71910=CARTESIAN_POINT ( 'NONE',  ( -72.65119488294536154, -291.0791912782864301, -206.3415606011172088 ) ) ;
#71912=CARTESIAN_POINT ( 'NONE',  ( 27.36219212280433055, -272.6237833571633473, -239.2376011013261916 ) ) ;
#71913=CARTESIAN_POINT ( 'NONE',  ( -113.4210998570117681, -295.4776246276126130, -280.9853841982642848 ) ) ;
#71914=CARTESIAN_POINT ( 'NONE',  ( -105.3381240462962722, -285.4110999573703111, -305.5449446909397011 ) ) ;
#71915=CARTESIAN_POINT ( 'NONE',  ( 13.14108632914916264, -286.6147167758442720, -217.5610405691734570 ) ) ;
#71916=CARTESIAN_POINT ( 'NONE',  ( 33.57026393535169007, -277.3354534249484118, -290.4622935678258386 ) ) ;
#71917=CARTESIAN_POINT ( 'NONE',  ( -12.48374081865526541, -292.7475294770085839, -340.7997187035144293 ) ) ;
#71918=CARTESIAN_POINT ( 'NONE',  ( -10.09641221913822129, -296.4516487380982426, -339.1773101233405328 ) ) ;
#71919=CARTESIAN_POINT ( 'NONE',  ( -39.18302286459971384, -275.8706939163810716, -343.7350918185940145 ) ) ;
#71922=CARTESIAN_POINT ( 'NONE',  ( -108.3571779278150160, -295.8393694218985956, -300.2067756596275103 ) ) ;
#71923=CARTESIAN_POINT ( 'NONE',  ( 2.094785200861719154, -290.4398222184229894, -333.4965107657784529 ) ) ;
#71925=CARTESIAN_POINT ( 'NONE',  ( -113.4697727941914422, -273.8642838345909922, -261.8449410113341855 ) ) ;
#71926=CARTESIAN_POINT ( 'NONE',  ( 2.495627169251863009, -287.2532947722501149, -209.0677250120993449 ) ) ;
#71928=CARTESIAN_POINT ( 'NONE',  ( -11.57700185046107499, -279.4382840174307603, -197.9934747404690825 ) ) ;
#71929=CARTESIAN_POINT ( 'NONE',  ( 28.02365960625705910, -294.7351142535849249, -310.9665138797749933 ) ) ;
#71930=CARTESIAN_POINT ( 'NONE',  ( -31.93890055105967107, -287.1243899591129320, -345.9847521395220724 ) ) ;
#71931=CARTESIAN_POINT ( 'NONE',  ( -47.62454736191332216, -295.5127642150984002, -346.6500906078986191 ) ) ;
#71932=CARTESIAN_POINT ( 'NONE',  ( 35.64232835602799554, -293.8547356705887523, -268.0332277545080046 ) ) ;
#71935=CARTESIAN_POINT ( 'NONE',  ( 4.780671393231641808, -288.1295972354226933, -206.6710476202246696 ) ) ;
#71936=CARTESIAN_POINT ( 'NONE',  ( 13.79469577742117181, -285.9094976428776249, -334.5364918783848793 ) ) ;
#71938=CARTESIAN_POINT ( 'NONE',  ( -50.91348084202865465, -279.2316788741146070, -194.6701703431777730 ) ) ;
#71939=CARTESIAN_POINT ( 'NONE',  ( -94.81413068156820145, -285.8888655477211955, -318.2876049841835311 ) ) ;
#71940=CARTESIAN_POINT ( 'NONE',  ( -113.0184284125890315, -282.9890047163514168, -281.3014110167351873 ) ) ;
#71941=CARTESIAN_POINT ( 'NONE',  ( 25.43995515728951062, -286.1743585002390660, -310.3583423453236492 ) ) ;
#71942=CARTESIAN_POINT ( 'NONE',  ( 22.55632473083532474, -278.0423500418750109, -316.7775556500084235 ) ) ;
#71943=CARTESIAN_POINT ( 'NONE',  ( -103.2259789066393694, -273.3111256698079501, -238.8754181093392788 ) ) ;
#71946=CARTESIAN_POINT ( 'NONE',  ( -109.0432837039744527, -278.3704622780569480, -284.1342045455916150 ) ) ;
#71947=CARTESIAN_POINT ( 'NONE',  ( -85.54518307666643295, -278.7128038947416258, -215.4037081136465304 ) ) ;
#71948=CARTESIAN_POINT ( 'NONE',  ( 23.37963922902225988, -276.0038610314780385, -223.4952015767635487 ) ) ;
#71949=CARTESIAN_POINT ( 'NONE',  ( -79.67848275044005391, -278.2889930618100607, -206.4570263846184162 ) ) ;
#71950=CARTESIAN_POINT ( 'NONE',  ( -100.0119297896911377, -246.0268988372215802, -332.0617019485725336 ) ) ;
#71952=CARTESIAN_POINT ( 'NONE',  ( -97.77916941543628582, -298.6065970111420143, -223.5861859380696899 ) ) ;
#71953=CARTESIAN_POINT ( 'NONE',  ( 31.95455697924148097, -283.6233781216988064, -236.9535640164627637 ) ) ;
#71956=CARTESIAN_POINT ( 'NONE',  ( -87.91765652325517522, -286.4041919975886685, -217.2923069180827440 ) ) ;
#71957=CARTESIAN_POINT ( 'NONE',  ( -77.99943868372949396, -287.2738242607385928, -206.1667077263731471 ) ) ;
#71958=CARTESIAN_POINT ( 'NONE',  ( 34.62057467902984342, -287.0701160298207810, -283.2189433421929152 ) ) ;
#71959=CARTESIAN_POINT ( 'NONE',  ( -114.2648508637497287, -284.1004888162801763, -267.1107478745750541 ) ) ;
#71960=CARTESIAN_POINT ( 'NONE',  ( 21.98409525709180556, -279.3430133537986535, -226.4434813437808884 ) ) ;
#71961=CARTESIAN_POINT ( 'NONE',  ( 5.417824719659231292, -288.4977835412642548, -209.6147155440238237 ) ) ;
#71962=CARTESIAN_POINT ( 'NONE',  ( -6.461383909828068539, -278.9451089280148608, -203.4361030857936612 ) ) ;
#71963=CARTESIAN_POINT ( 'NONE',  ( -96.47993366906230506, -279.2596039383150242, -314.0160555217643150 ) ) ;
#71964=CARTESIAN_POINT ( 'NONE',  ( 30.33739946726818815, -276.4144734333676183, -298.0189885474565017 ) ) ;
#71965=CARTESIAN_POINT ( 'NONE',  ( 16.39641102352779001, -287.1045198474900531, -325.0262930092932834 ) ) ;
#71967=CARTESIAN_POINT ( 'NONE',  ( -79.06345468238039587, -284.4024513556360603, -334.8859505441761257 ) ) ;
#71968=CARTESIAN_POINT ( 'NONE',  ( 11.45841264937041082, -282.8888217031168324, -329.9117917402192006 ) ) ;
#71969=ORIENTED_EDGE ( 'NONE', *, *, #60435, .T. ) ;
#71972=CARTESIAN_POINT ( 'NONE',  ( -41.66599189590501595, -290.9664623462520012, -346.0154262564238365 ) ) ;
#71973=CARTESIAN_POINT ( 'NONE',  ( -113.8750804876521130, -289.2622826738865456, -268.3508496036086513 ) ) ;
#71974=CARTESIAN_POINT ( 'NONE',  ( -46.19537902311201805, -272.9958229657343622, -197.6629693275739612 ) ) ;
#71975=CARTESIAN_POINT ( 'NONE',  ( 35.35896607655254797, -292.5826404289562674, -245.1414319223741529 ) ) ;
#71976=CARTESIAN_POINT ( 'NONE',  ( -110.8155546239507601, -288.9495792697245520, -276.6701798364307479 ) ) ;
#71977=CARTESIAN_POINT ( 'NONE',  ( 21.81708044103580235, -291.1760203637315954, -225.8840149151220942 ) ) ;
#71978=CARTESIAN_POINT ( 'NONE',  ( 12.43630700787172749, -289.5455572973409062, -324.3679410442289281 ) ) ;
#71979=CARTESIAN_POINT ( 'NONE',  ( -54.42813229853333468, -291.7662352645558599, -345.3683826091709648 ) ) ;
#71980=CARTESIAN_POINT ( 'NONE',  ( -48.54443258265927597, -291.1948055562469335, -344.5722688021063504 ) ) ;
#71981=CARTESIAN_POINT ( 'NONE',  ( -93.32835501897923791, -289.2489799189719974, -220.2061291768349065 ) ) ;
#71983=CARTESIAN_POINT ( 'NONE',  ( -40.01351806051105342, -294.0187654585725454, -195.3961402325638517 ) ) ;
#71984=CARTESIAN_POINT ( 'NONE',  ( -110.5448710370901040, -285.5219295795045582, -268.1921974500549481 ) ) ;
#71985=CARTESIAN_POINT ( 'NONE',  ( 7.730752589637974737, -294.6656197581439187, -210.1421827852705633 ) ) ;
#71988=CARTESIAN_POINT ( 'NONE',  ( -92.94891957850609288, -275.2389527599934809, -219.4869315965473220 ) ) ;
#71989=CARTESIAN_POINT ( 'NONE',  ( 33.11219503982915313, -281.0093767456083924, -290.0804075981376968 ) ) ;
#71990=CARTESIAN_POINT ( 'NONE',  ( -32.02876435720155257, -280.9849457034831062, -345.1727037359891028 ) ) ;
#71991=CARTESIAN_POINT ( 'NONE',  ( -53.26578666536293127, -294.4483887895736416, -345.5859034630552173 ) ) ;
#71992=CARTESIAN_POINT ( 'NONE',  ( 5.785153532394141429, -272.8850983219649606, -210.1475440307942222 ) ) ;
#71993=CARTESIAN_POINT ( 'NONE',  ( -97.26648212413840611, -276.0247988262237300, -314.5450866642938763 ) ) ;
#71994=CARTESIAN_POINT ( 'NONE',  ( -63.26901759104931955, -299.0224993134086162, -201.5394178659348086 ) ) ;
#71995=CARTESIAN_POINT ( 'NONE',  ( -29.87824091759911127, -272.7196098822664680, -194.3157166157376992 ) ) ;
#71996=CARTESIAN_POINT ( 'NONE',  ( 35.87970261879645761, -294.8748380253817913, -262.5212469478725552 ) ) ;
#71998=CARTESIAN_POINT ( 'NONE',  ( 10.40461484679384263, -295.1757085248730164, -325.7947822380005505 ) ) ;
#72000=CARTESIAN_POINT ( 'NONE',  ( -18.56692111267556200, -284.3127753800040409, -197.3283248519107929 ) ) ;
#72001=CARTESIAN_POINT ( 'NONE',  ( -96.10032005947223865, -297.1595038245295086, -227.0222975241949541 ) ) ;
#72002=CARTESIAN_POINT ( 'NONE',  ( -99.34424074211752043, -285.1597386703469397, -224.6150375898039329 ) ) ;
#72003=CARTESIAN_POINT ( 'NONE',  ( 32.69455555656799106, -286.8089138047854476, -238.2849010246100363 ) ) ;
#72004=CARTESIAN_POINT ( 'NONE',  ( 25.16186041069929047, -296.0986839325759092, -312.4528240888232062 ) ) ;
#72005=CARTESIAN_POINT ( 'NONE',  ( 35.08894215874857991, -291.3097428907472590, -251.5507355454824108 ) ) ;
#72007=CARTESIAN_POINT ( 'NONE',  ( -94.83416476701385989, -278.4414727312155833, -219.3829331338753263 ) ) ;
#72009=CARTESIAN_POINT ( 'NONE',  ( -37.30987171927208834, -283.5523547857346784, -195.3611179825600175 ) ) ;
#72011=CARTESIAN_POINT ( 'NONE',  ( 25.29754418281599371, -285.8228712985219317, -232.1059800730079132 ) ) ;
#72014=CARTESIAN_POINT ( 'NONE',  ( -111.0395096149018315, -298.1016273590528272, -274.2435515210606809 ) ) ;
#72015=CARTESIAN_POINT ( 'NONE',  ( -25.50490493817391169, -281.6254462949252115, -194.8727309868217503 ) ) ;
#72016=CARTESIAN_POINT ( 'NONE',  ( -73.83245331181514359, -293.5539221253186497, -336.3500708814008817 ) ) ;
#72017=CARTESIAN_POINT ( 'NONE',  ( 35.03278949103064832, -281.4214001322674221, -260.4493991356154083 ) ) ;
#72018=CARTESIAN_POINT ( 'NONE',  ( -81.86997073787379975, -295.8067354970518181, -333.2452900623168830 ) ) ;
#72019=CARTESIAN_POINT ( 'NONE',  ( -101.2383276382620636, -274.4748131363380139, -233.7538662865325136 ) ) ;
#72020=CARTESIAN_POINT ( 'NONE',  ( -66.60618896100223196, -281.6689944610478733, -201.3061373944859156 ) ) ;
#72021=CARTESIAN_POINT ( 'NONE',  ( -109.5056735946826336, -295.7750097042693369, -257.8803575086465116 ) ) ;
#72024=CARTESIAN_POINT ( 'NONE',  ( -34.76506622459292828, -284.9995455357266110, -344.9741545967229399 ) ) ;
#72026=CARTESIAN_POINT ( 'NONE',  ( -69.85430415644619018, -283.1237833571632336, -202.7746430608542312 ) ) ;
#72027=CARTESIAN_POINT ( 'NONE',  ( 32.41078021772341344, -274.3346903715184908, -238.0047266940846953 ) ) ;
#72028=CARTESIAN_POINT ( 'NONE',  ( -28.10424422201742800, -292.0058468812596857, -197.8971842642352783 ) ) ;
#72029=CARTESIAN_POINT ( 'NONE',  ( 28.78165832251644218, -283.5103397503215774, -303.0101868851732547 ) ) ;
#72031=CARTESIAN_POINT ( 'NONE',  ( 35.41089927456891218, -276.9896402802463058, -257.8966782738378356 ) ) ;
#72032=CARTESIAN_POINT ( 'NONE',  ( 32.83718764427325709, -283.5356054391248222, -300.1837324166258441 ) ) ;
#72033=CARTESIAN_POINT ( 'NONE',  ( 19.65070171970234014, -280.9981525836967649, -316.6302118931899940 ) ) ;
#72034=CARTESIAN_POINT ( 'NONE',  ( -109.9141424287481215, -280.7961214337716456, -251.3833419120509802 ) ) ;
#72035=CARTESIAN_POINT ( 'NONE',  ( -30.48458194015535838, -298.1357836350427419, -193.3611176790317074 ) ) ;
#72036=CARTESIAN_POINT ( 'NONE',  ( 39.55446787631457539, -275.3239508089454830, -265.4418929110120189 ) ) ;
#72037=CARTESIAN_POINT ( 'NONE',  ( 35.35080722273567488, -295.2641107008909103, -254.2675017003034839 ) ) ;
#72038=DIRECTION ( 'NONE',  ( 0.000000000000000000, 0.000000000000000000, 1.000000000000000000 ) ) ;
#72040=CARTESIAN_POINT ( 'NONE',  ( -5.050829660353836736, -292.7712104210492612, -338.9144308581992959 ) ) ;
#72041=CARTESIAN_POINT ( 'NONE',  ( -46.18001305785128352, -273.4446554223143835, -197.8361383814520309 ) ) ;
#72042=CARTESIAN_POINT ( 'NONE',  ( -14.09625302340793418, -293.8683044725487434, -197.6258270216233939 ) ) ;
#72043=CARTESIAN_POINT ( 'NONE',  ( 21.27581636871892101, -283.4090924074130839, -223.5744983911110353 ) ) ;
#72044=CARTESIAN_POINT ( 'NONE',  ( -58.84201449618048230, -292.9851042784021615, -196.8373449585159278 ) ) ;
#72045=CARTESIAN_POINT ( 'NONE',  ( -34.48307862508264776, -291.0164376147766347, -345.1906619236081042 ) ) ;
#72046=CARTESIAN_POINT ( 'NONE',  ( -88.36366393943762887, -275.7689532936446426, -325.1040411158176653 ) ) ;
#72047=CARTESIAN_POINT ( 'NONE',  ( -35.04926656989797351, -278.9432927561168185, -344.7658150714715930 ) ) ;
#72048=CARTESIAN_POINT ( 'NONE',  ( 15.31800204115145547, -292.3814875157432311, -323.0479202010999416 ) ) ;
#72049=CARTESIAN_POINT ( 'NONE',  ( 14.91893594893046426, -284.1850968029752380, -325.2166682538226610 ) ) ;
#72050=CARTESIAN_POINT ( 'NONE',  ( -109.9163088430971129, -283.6084530073849237, -260.0096811946550019 ) ) ;
#72052=CARTESIAN_POINT ( 'NONE',  ( 7.803703418024110050, -282.0829779783930462, -327.8188973778915738 ) ) ;
#72053=CARTESIAN_POINT ( 'NONE',  ( -8.988225947576655273, -281.4941050074010036, -199.1040270246605814 ) ) ;
#72054=CARTESIAN_POINT ( 'NONE',  ( -106.6529233668657497, -282.9271153624624162, -302.9795644600513356 ) ) ;
#72055=CARTESIAN_POINT ( 'NONE',  ( -108.2997405067442429, -279.8667756047477724, -241.0732925599855321 ) ) ;
#72056=CARTESIAN_POINT ( 'NONE',  ( -25.85505919037385425, -278.4285036815351759, -345.7982761425820968 ) ) ;
#72057=CARTESIAN_POINT ( 'NONE',  ( -82.08285599513421005, -298.1948066931273615, -326.5171145203363494 ) ) ;
#72059=CARTESIAN_POINT ( 'NONE',  ( -94.32598840690097575, -275.2254758088072890, -221.8354602036058338 ) ) ;
#72060=CARTESIAN_POINT ( 'NONE',  ( -93.99100174651738371, -275.8955222071638218, -318.9687658516154443 ) ) ;
#72061=CARTESIAN_POINT ( 'NONE',  ( -105.1106540324819036, -292.7619993617021805, -235.8743658751812973 ) ) ;
#72062=CARTESIAN_POINT ( 'NONE',  ( 24.50908012278991777, -293.4393963967647210, -309.4225019919180681 ) ) ;
#72063=CARTESIAN_POINT ( 'NONE',  ( -75.63849464279904566, -289.0566755653645714, -337.0910395556628032 ) ) ;
#72065=CARTESIAN_POINT ( 'NONE',  ( 38.23108079138106064, -292.2691119007565135, -281.6465544832571481 ) ) ;
#72066=CARTESIAN_POINT ( 'NONE',  ( -19.60405935796048027, -284.6839469424128879, -198.7244198946049210 ) ) ;
#72067=CARTESIAN_POINT ( 'NONE',  ( -58.02137488133270438, -293.6427136461132363, -199.0106616299309223 ) ) ;
#72068=CARTESIAN_POINT ( 'NONE',  ( -35.90068164768727144, -284.5504271968976582, -196.6818724648418026 ) ) ;
#72069=CARTESIAN_POINT ( 'NONE',  ( 14.28293525582184564, -283.6235352786957264, -322.7409180634737709 ) ) ;
#72070=CARTESIAN_POINT ( 'NONE',  ( -59.94651908012836117, -290.2793647248366824, -343.7221592277097102 ) ) ;
#72071=CARTESIAN_POINT ( 'NONE',  ( 31.12577768059959737, -281.7029552731623880, -244.7171264559154338 ) ) ;
#72072=CARTESIAN_POINT ( 'NONE',  ( 19.22604116101428673, -293.0537110175874318, -322.0920100187227604 ) ) ;
#72073=CARTESIAN_POINT ( 'NONE',  ( -23.33132271493577647, -289.6803567608358208, -345.9655546087703328 ) ) ;
#72075=CARTESIAN_POINT ( 'NONE',  ( -82.81122626075774917, -290.1479625329168925, -332.4259961048541072 ) ) ;
#72076=CARTESIAN_POINT ( 'NONE',  ( -108.3660055645780744, -284.9420133606111563, -253.4387241064036118 ) ) ;
#72079=CARTESIAN_POINT ( 'NONE',  ( 20.44122463352771035, -296.0838475890648169, -319.3655982784746925 ) ) ;
#72080=CARTESIAN_POINT ( 'NONE',  ( -104.1802850471923989, -294.7500243254506245, -307.6971628235469893 ) ) ;
#72081=CARTESIAN_POINT ( 'NONE',  ( -96.58902260927307282, -278.2114451816100882, -227.3127355810333938 ) ) ;
#72082=CARTESIAN_POINT ( 'NONE',  ( -78.80311177904566478, -273.0169954203856832, -205.5500213474510929 ) ) ;
#72083=CARTESIAN_POINT ( 'NONE',  ( -80.57704693125474193, -294.1303770366412778, -330.0386894608332113 ) ) ;
#72084=CARTESIAN_POINT ( 'NONE',  ( 31.22514465699807573, -277.6820633777243188, -298.3644491461026291 ) ) ;
#72085=CARTESIAN_POINT ( 'NONE',  ( -108.3715727417624777, -270.9747709077365130, -248.6069281272188505 ) ) ;
#72086=CARTESIAN_POINT ( 'NONE',  ( 31.91983378390802173, -295.0804446200519919, -294.8026977361891454 ) ) ;
#72087=CARTESIAN_POINT ( 'NONE',  ( -71.06079061321462120, -296.5877362488466815, -335.4693154410733200 ) ) ;
#72088=CARTESIAN_POINT ( 'NONE',  ( -108.1158907659633996, -294.8793984399376882, -245.0423035400979472 ) ) ;
#72089=CARTESIAN_POINT ( 'NONE',  ( 53.42971810148159761, -299.8120856905852065, -193.4532684622509180 ) ) ;
#72090=CARTESIAN_POINT ( 'NONE',  ( -33.97572615395107931, -276.0946628083879659, -195.4366835832176150 ) ) ;
#72091=CARTESIAN_POINT ( 'NONE',  ( -74.82606945250284980, -290.5056965738940562, -333.2911152893400413 ) ) ;
#72092=CARTESIAN_POINT ( 'NONE',  ( -108.0234513516876405, -273.4334574445227872, -239.8352910743383575 ) ) ;
#72093=CARTESIAN_POINT ( 'NONE',  ( -26.19999564173576800, -295.2396752348956284, -342.5272451326647456 ) ) ;
#72095=CARTESIAN_POINT ( 'NONE',  ( -112.5703135575944316, -280.5878421184739864, -265.9950531963937692 ) ) ;
#72096=CARTESIAN_POINT ( 'NONE',  ( -69.73821498184940992, -278.3193582752171551, -201.0376299117948804 ) ) ;
#72097=CARTESIAN_POINT ( 'NONE',  ( -47.25145265047196119, -282.5235153986121759, -346.6179838461253553 ) ) ;
#72098=CARTESIAN_POINT ( 'NONE',  ( 22.68399703883054030, -274.2558517652779528, -222.2753977917737416 ) ) ;
#72099=CARTESIAN_POINT ( 'NONE',  ( -84.06021005979886240, -277.8224186699837333, -210.0961750148686349 ) ) ;
#72100=CARTESIAN_POINT ( 'NONE',  ( -36.74099793837045524, -278.0595291237798392, -195.1841118836794067 ) ) ;
#72101=CARTESIAN_POINT ( 'NONE',  ( -34.43878961313275511, -296.7740619526214232, -196.8686294547052569 ) ) ;
#72102=CARTESIAN_POINT ( 'NONE',  ( 37.17243969616534827, -277.4372861856307395, -261.4024133701462915 ) ) ;
#72104=CARTESIAN_POINT ( 'NONE',  ( -9.103671700846375003, -290.4396919338562952, -200.4968169823320352 ) ) ;
#72105=CARTESIAN_POINT ( 'NONE',  ( -69.62316028454603156, -291.6388648731768285, -200.4403581354582968 ) ) ;
#72106=CARTESIAN_POINT ( 'NONE',  ( -68.11731033356453224, -275.6491723209145448, -201.7694409521948558 ) ) ;
#72107=CARTESIAN_POINT ( 'NONE',  ( -109.8677007266892076, -270.7998507818898588, -251.0577745248691599 ) ) ;
#72109=CARTESIAN_POINT ( 'NONE',  ( -113.3261760821276596, -283.8968945801153723, -258.5861112596620046 ) ) ;
#72111=CARTESIAN_POINT ( 'NONE',  ( -86.78430732134359005, -283.3648139544016544, -213.8977631919859448 ) ) ;
#72113=CARTESIAN_POINT ( 'NONE',  ( -12.10936487513805560, -291.1827287707544656, -201.3833634643218602 ) ) ;
#72114=CARTESIAN_POINT ( 'NONE',  ( -52.31531814145177606, -283.9979545309563491, -197.6517221586202595 ) ) ;
#72117=CARTESIAN_POINT ( 'NONE',  ( 22.91862670923142886, -292.1613886544911907, -315.0119148497878996 ) ) ;
#72118=CARTESIAN_POINT ( 'NONE',  ( -113.1287578992756266, -283.1442229707908496, -261.4712571083671264 ) ) ;
#72119=CARTESIAN_POINT ( 'NONE',  ( -95.06616654416247059, -279.5097037708815151, -316.3631023532406630 ) ) ;
#72120=CARTESIAN_POINT ( 'NONE',  ( -108.9263851094585362, -285.4085708248432525, -297.7786406815976079 ) ) ;
#72121=CARTESIAN_POINT ( 'NONE',  ( 33.38856281973362883, -287.3131462519596084, -252.2488282641054980 ) ) ;
#72122=CARTESIAN_POINT ( 'NONE',  ( -85.47706236587302442, -279.1580606253975247, -326.0915339580321870 ) ) ;
#72123=CARTESIAN_POINT ( 'NONE',  ( -100.9572441311622981, -279.8487660301154847, -234.2271410665883877 ) ) ;
#72124=CARTESIAN_POINT ( 'NONE',  ( -21.35796284116707966, -288.2360637772588916, -196.7205928480166790 ) ) ;
#72126=CARTESIAN_POINT ( 'NONE',  ( 7.991229253068932614, -298.4383658456491730, -193.3623461297880226 ) ) ;
#72127=CARTESIAN_POINT ( 'NONE',  ( -20.73952784644652070, -290.8178684932008196, -343.1362145134649495 ) ) ;
#72129=CARTESIAN_POINT ( 'NONE',  ( -115.3430155898818299, -287.2662352645559167, -252.5904736702033517 ) ) ;
#72131=CARTESIAN_POINT ( 'NONE',  ( 20.74446902344014632, -292.6238628041645029, -319.6808642372171789 ) ) ;
#72132=CARTESIAN_POINT ( 'NONE',  ( 11.58000868160295127, -288.2653677199208460, -215.1801947130151405 ) ) ;
#72133=CARTESIAN_POINT ( 'NONE',  ( -19.30906643256497546, -282.0473460733831530, -198.5251132865508623 ) ) ;
#72134=CARTESIAN_POINT ( 'NONE',  ( 25.05338678105322359, -288.3889508617324395, -226.2312038807338013 ) ) ;
#72135=CARTESIAN_POINT ( 'NONE',  ( 32.42209717841763705, -289.2710504435426628, -301.7667043778193943 ) ) ;
#72136=CARTESIAN_POINT ( 'NONE',  ( -67.33667069520981840, -285.4456307096435808, -339.1158932400369395 ) ) ;
#72137=CARTESIAN_POINT ( 'NONE',  ( -109.7360357469265182, -278.3857713052277632, -296.7479835589050481 ) ) ;
#72139=CARTESIAN_POINT ( 'NONE',  ( 16.51762841623082068, -292.3741761567443973, -323.4306708985980663 ) ) ;
#72140=CARTESIAN_POINT ( 'NONE',  ( 19.16160386343882038, -280.6729170352049891, -218.0507304620034006 ) ) ;
#72141=CARTESIAN_POINT ( 'NONE',  ( -86.13965362379038027, -275.2278293405495333, -214.3495325486017293 ) ) ;
#72142=CARTESIAN_POINT ( 'NONE',  ( 10.64812456238590066, -290.9090924074130839, -330.4860931364851808 ) ) ;
#72143=CARTESIAN_POINT ( 'NONE',  ( -5.517966667665570313, -272.7049106162600651, -201.3594947734044638 ) ) ;
#72145=CARTESIAN_POINT ( 'NONE',  ( -22.17551659206192838, -279.7592038649978576, -198.8391152777686557 ) ) ;
#72146=CARTESIAN_POINT ( 'NONE',  ( 37.55390969369304344, -276.5542630946214331, -254.2163673217129372 ) ) ;
#72147=CARTESIAN_POINT ( 'NONE',  ( -82.31847732346159319, -298.8501617088954276, -212.0516574874254445 ) ) ;
#72148=CARTESIAN_POINT ( 'NONE',  ( -13.50640716079615267, -281.8088008064682981, -343.3316532805359316 ) ) ;
#72149=CARTESIAN_POINT ( 'NONE',  ( -93.33763987949404850, -292.9924453883014621, -221.9624739252059271 ) ) ;
#72150=CARTESIAN_POINT ( 'NONE',  ( -92.60614567709042433, -274.8769020882753011, -217.8798799866181923 ) ) ;
#72151=CARTESIAN_POINT ( 'NONE',  ( -20.63312189431888299, -299.4620382776674319, -193.7548524899362974 ) ) ;
#72152=CARTESIAN_POINT ( 'NONE',  ( 36.71857844773398227, -295.4142531729041821, -259.6324850765803376 ) ) ;
#72153=CARTESIAN_POINT ( 'NONE',  ( -106.9278959403439870, -282.1911459951321035, -298.0302777590979986 ) ) ;
#72154=CARTESIAN_POINT ( 'NONE',  ( -101.6639569753313310, -290.7760345106847808, -227.9760924588899798 ) ) ;
#72155=CARTESIAN_POINT ( 'NONE',  ( -93.23337476386113565, -271.2636306261364325, -220.8841788005876197 ) ) ;
#72156=CARTESIAN_POINT ( 'NONE',  ( -40.80076927130045306, -287.6095817238835366, -194.1880173347707341 ) ) ;
#72157=CARTESIAN_POINT ( 'NONE',  ( -75.12719568111137391, -290.4565565351510941, -207.4808241759919269 ) ) ;
#72158=VERTEX_POINT ( 'NONE', #23027 ) ;
#72159=CARTESIAN_POINT ( 'NONE',  ( -93.17475775510396829, -288.4093747830734742, -322.6032448801970531 ) ) ;
#72160=CARTESIAN_POINT ( 'NONE',  ( -61.26594495987933442, -289.0382953878480521, -339.3518274728278357 ) ) ;
#72162=CARTESIAN_POINT ( 'NONE',  ( -64.45083892249839153, -286.7861564909559320, -198.6072883698452927 ) ) ;
#72163=CARTESIAN_POINT ( 'NONE',  ( -93.61961422051079751, -278.2258150813962629, -316.9090201112134650 ) ) ;
#72164=CARTESIAN_POINT ( 'NONE',  ( 10.93491539985237893, -291.6222251664050304, -210.7036837983360726 ) ) ;
#72165=CARTESIAN_POINT ( 'NONE',  ( -95.25249656028125855, -284.5183881449053160, -320.9541258333605356 ) ) ;
#72166=CARTESIAN_POINT ( 'NONE',  ( -113.7991315765020772, -284.9973273255151298, -261.4165404187135664 ) ) ;
#72167=CARTESIAN_POINT ( 'NONE',  ( -62.32016810646861416, -280.0515117301268901, -201.6916843282011484 ) ) ;
#72168=CARTESIAN_POINT ( 'NONE',  ( -12.65737504837112404, -91.72627791072594050, -360.1682197548814202 ) ) ;
#72169=CARTESIAN_POINT ( 'NONE',  ( 137.7092865063222575, 180.7388654737660829, -240.7682804503873797 ) ) ;
#72170=CARTESIAN_POINT ( 'NONE',  ( 44.12421593066579106, 11.81245027319820196, -328.6256852122805867 ) ) ;
#72171=CARTESIAN_POINT ( 'NONE',  ( -83.28406724776048975, -272.6009407282153916, -213.4234272157443115 ) ) ;
#72172=CARTESIAN_POINT ( 'NONE',  ( 21.73841949090026660, -273.8669598924385014, -226.9587500736770096 ) ) ;
#72173=CARTESIAN_POINT ( 'NONE',  ( -61.57813148803720082, -294.8663075684704040, -343.4381965951935740 ) ) ;
#72174=CARTESIAN_POINT ( 'NONE',  ( -92.86534849868182562, -239.6190322135574604, -339.0248232835550652 ) ) ;
#72175=CARTESIAN_POINT ( 'NONE',  ( -21.44083504604207135, -272.9367847985587332, -195.5248917209902118 ) ) ;
#72176=CARTESIAN_POINT ( 'NONE',  ( -36.48891269409420346, -299.9233529725826770, -196.1256365755298248 ) ) ;
#72177=CARTESIAN_POINT ( 'NONE',  ( -3.121925690105149975, -289.9057000701648690, -335.4578648123214180 ) ) ;
#72179=CARTESIAN_POINT ( 'NONE',  ( 21.19602096002916269, -295.1648322703576923, -320.0215189419722037 ) ) ;
#72180=CARTESIAN_POINT ( 'NONE',  ( -60.00366422690770918, -286.2427252602014960, -200.9030455593933482 ) ) ;
#72181=CARTESIAN_POINT ( 'NONE',  ( -100.9444605425184704, -272.0403866702864093, -227.4159127912577958 ) ) ;
#72182=CARTESIAN_POINT ( 'NONE',  ( 38.65834229362575059, -294.4968572137112801, -281.6815584508277652 ) ) ;
#72183=CARTESIAN_POINT ( 'NONE',  ( -105.9000167581246927, -296.5931517407428828, -305.3967080702572616 ) ) ;
#72184=CARTESIAN_POINT ( 'NONE',  ( -108.7110157719450001, -290.9212379986113319, -255.0176897782157539 ) ) ;
#72186=CARTESIAN_POINT ( 'NONE',  ( -84.92079890458373370, -275.3217943752956671, -211.6623653999179453 ) ) ;
#72187=CARTESIAN_POINT ( 'NONE',  ( 34.82171282160243919, -274.6748853042140013, -296.2166109889252539 ) ) ;
#72189=CARTESIAN_POINT ( 'NONE',  ( -109.6810496182796300, -277.7268502464187918, -296.7190168683673619 ) ) ;
#72190=CARTESIAN_POINT ( 'NONE',  ( 36.14881875116507359, -274.0401164478188321, -277.1127140063403544 ) ) ;
#72191=CARTESIAN_POINT ( 'NONE',  ( -64.69684565372234886, -274.7660610395514595, -202.3334482827306715 ) ) ;
#72192=CARTESIAN_POINT ( 'NONE',  ( 25.47149148025363985, -275.9759358689927922, -232.6077533692073871 ) ) ;
#72193=CARTESIAN_POINT ( 'NONE',  ( 35.60663071739295304, -277.0398496886527369, -248.9050339979837361 ) ) ;
#72194=CARTESIAN_POINT ( 'NONE',  ( 32.64702206594044043, -273.9359372376582655, -298.4299030441207492 ) ) ;
#72195=CARTESIAN_POINT ( 'NONE',  ( -5.489605120973596541, -295.2731202430690587, -336.1726441367379152 ) ) ;
#72196=CARTESIAN_POINT ( 'NONE',  ( -35.65516140443621396, -293.6053406829528285, -343.9436173441469009 ) ) ;
#72198=CARTESIAN_POINT ( 'NONE',  ( -82.20805887752608498, -279.9503500644127030, -207.8588239795570587 ) ) ;
#72199=CARTESIAN_POINT ( 'NONE',  ( 0.8732352476282526643, -276.6939008672684395, -332.6187364180840405 ) ) ;
#72200=CARTESIAN_POINT ( 'NONE',  ( -46.43019579271401653, -284.6239346561618504, -194.3960107384411629 ) ) ;
#72201=CARTESIAN_POINT ( 'NONE',  ( -71.22427780113663687, -297.4985909101912966, -337.4580580063670254 ) ) ;
#72203=CARTESIAN_POINT ( 'NONE',  ( 35.71455348921347195, -286.6864663648976261, -265.5863291493671454 ) ) ;
#72205=CARTESIAN_POINT ( 'NONE',  ( -69.71460270213881927, -275.7241295772534500, -336.9331624954579638 ) ) ;
#72206=CARTESIAN_POINT ( 'NONE',  ( -110.9816351847938307, -277.1234559487222668, -270.6221747619007942 ) ) ;
#72207=CARTESIAN_POINT ( 'NONE',  ( -111.9586348641968243, -286.4487947236958689, -278.4235455609854171 ) ) ;
#72208=CARTESIAN_POINT ( 'NONE',  ( -32.37846152274660483, -278.1934021981566616, -343.6404262525761055 ) ) ;
#72210=CARTESIAN_POINT ( 'NONE',  ( 23.71430784749315279, -274.5649275561231661, -315.9528311257732867 ) ) ;
#72211=CARTESIAN_POINT ( 'NONE',  ( 35.12045750345512118, -276.0764425751135036, -260.7108133468422011 ) ) ;
#72212=CARTESIAN_POINT ( 'NONE',  ( 26.28556427364415526, -283.0143621062061356, -230.2436344752042032 ) ) ;
#72214=CARTESIAN_POINT ( 'NONE',  ( 9.357531784683576603, -290.3366721901008987, -329.8288423934346838 ) ) ;
#72215=CARTESIAN_POINT ( 'NONE',  ( 13.21780444310662261, -290.7583603155152332, -214.8954347324663274 ) ) ;
#72217=CARTESIAN_POINT ( 'NONE',  ( -107.6635277046676578, -271.5199248403631032, -248.8308006682090365 ) ) ;
#72218=CARTESIAN_POINT ( 'NONE',  ( -108.5739573580552957, -288.9641819618393583, -249.4155292926967320 ) ) ;
#72219=CARTESIAN_POINT ( 'NONE',  ( -92.95696114837319612, -243.2523998898738569, -344.1903318997441374 ) ) ;
#72221=CARTESIAN_POINT ( 'NONE',  ( -111.8921524909754339, -288.8266219521386233, -286.6380282534744879 ) ) ;
#72222=CARTESIAN_POINT ( 'NONE',  ( -109.7606390010757025, -285.9668556064560789, -284.5715968414907024 ) ) ;
#72223=CARTESIAN_POINT ( 'NONE',  ( -113.3273347366348816, -282.7970378597454442, -269.9644513511321406 ) ) ;
#72225=CARTESIAN_POINT ( 'NONE',  ( 12.32765385669209302, -283.7694257046418329, -324.6596464212620390 ) ) ;
#72226=CARTESIAN_POINT ( 'NONE',  ( -100.5354780182555459, -284.8501155841900072, -307.2277446602610098 ) ) ;
#72227=CARTESIAN_POINT ( 'NONE',  ( -103.1853014058950606, -293.0174815337820178, -233.7137855962563719 ) ) ;
#72228=CARTESIAN_POINT ( 'NONE',  ( 7.219291916388593577, -274.9740221839773540, -207.5257884956481576 ) ) ;
#72229=CARTESIAN_POINT ( 'NONE',  ( -110.9095401712133935, -288.8516815247767227, -253.1249027969321048 ) ) ;
#72230=CARTESIAN_POINT ( 'NONE',  ( -87.09519316048870508, -277.7227055379217973, -329.1981338466251827 ) ) ;
#72231=CARTESIAN_POINT ( 'NONE',  ( -12.43620591708766909, -296.7066756333763919, -340.7829283047855711 ) ) ;
#72233=CARTESIAN_POINT ( 'NONE',  ( -95.95921662488163406, -298.4090924074130271, -317.1477375740089997 ) ) ;
#72234=CARTESIAN_POINT ( 'NONE',  ( -93.81167255414798944, -282.5740673866115458, -317.3971222088090371 ) ) ;
#72235=CARTESIAN_POINT ( 'NONE',  ( -94.36808371056892497, -277.2268040624016407, -221.6280328345879980 ) ) ;
#72236=CARTESIAN_POINT ( 'NONE',  ( -93.62070480235979630, -271.7395035847036411, -218.8114385640503201 ) ) ;
#72237=CARTESIAN_POINT ( 'NONE',  ( 22.54457857065109039, -275.4856188734532907, -312.3708708256971249 ) ) ;
#72238=CARTESIAN_POINT ( 'NONE',  ( -65.61065908443198680, -293.1957805189775286, -202.2918073840752982 ) ) ;
#72239=CARTESIAN_POINT ( 'NONE',  ( 34.94425714589072385, -294.3378254519152506, -258.5291048010317354 ) ) ;
#72240=CARTESIAN_POINT ( 'NONE',  ( 15.15256291725693139, -295.6446606146163276, -326.0176595489072611 ) ) ;
#72241=CARTESIAN_POINT ( 'NONE',  ( -103.7177047210294774, -296.7967053436346987, -239.8548220827740352 ) ) ;
#72242=CARTESIAN_POINT ( 'NONE',  ( -34.47676895978258926, -291.0164376166588340, -345.3573223174328177 ) ) ;
#72243=CARTESIAN_POINT ( 'NONE',  ( -24.53149152632248686, -283.0598036046549737, -346.3421632552261826 ) ) ;
#72244=CARTESIAN_POINT ( 'NONE',  ( -46.70449181843956410, -272.0740742925664222, -195.1770531096858861 ) ) ;
#72245=CARTESIAN_POINT ( 'NONE',  ( 39.60421368790518670, -287.4362975898073387, -274.4250517750303402 ) ) ;
#72246=CARTESIAN_POINT ( 'NONE',  ( -88.19814173176044392, -279.7483649707896234, -325.0005647948572118 ) ) ;
#72247=CARTESIAN_POINT ( 'NONE',  ( -62.63291473737278636, -284.7736471099571531, -201.5774035098777972 ) ) ;
#72248=CARTESIAN_POINT ( 'NONE',  ( -0.2914747910911555939, -286.5597075694872728, -335.6293159690200696 ) ) ;
#72249=CARTESIAN_POINT ( 'NONE',  ( 168.1488725781630649, 234.1813984995739588, -193.4213935641190858 ) ) ;
#72250=CARTESIAN_POINT ( 'NONE',  ( -107.8221751442056444, -283.8051593440850979, -289.6565123486637390 ) ) ;
#72251=CARTESIAN_POINT ( 'NONE',  ( 21.65503192903580754, -282.0969594670625611, -221.5001486240920769 ) ) ;
#72252=CARTESIAN_POINT ( 'NONE',  ( -9.659396615061330849, -287.7579253121039642, -341.9607708109615487 ) ) ;
#72253=CARTESIAN_POINT ( 'NONE',  ( -69.64200290103747193, -281.2341882915895326, -201.3314374808650769 ) ) ;
#72254=CARTESIAN_POINT ( 'NONE',  ( -109.1491771156735240, -280.2048636172129932, -243.8076120735747168 ) ) ;
#72255=CARTESIAN_POINT ( 'NONE',  ( -85.48258965898659767, -279.1974590404680612, -215.4843946869900151 ) ) ;
#72256=CARTESIAN_POINT ( 'NONE',  ( -57.32568297988208883, -275.7730335748682364, -198.3872028591245567 ) ) ;
#72257=CARTESIAN_POINT ( 'NONE',  ( 38.32523786283130107, -293.3737380188479733, -256.0952673216502262 ) ) ;
#72258=CARTESIAN_POINT ( 'NONE',  ( 34.66194084949533760, -285.8287690258733846, -290.2331922916596909 ) ) ;
#72259=CARTESIAN_POINT ( 'NONE',  ( 8.354722956675544765, -294.2656520259033073, -209.3175969661433271 ) ) ;
#72260=CARTESIAN_POINT ( 'NONE',  ( -93.32732666391014220, -294.8025412396413572, -317.7074719879774989 ) ) ;
#72261=CARTESIAN_POINT ( 'NONE',  ( -36.14635901347068625, -284.9572025038203833, -344.7915241410474891 ) ) ;
#72262=CARTESIAN_POINT ( 'NONE',  ( -53.15809115742599289, -294.9271576280351610, -341.7007697881484205 ) ) ;
#72263=CARTESIAN_POINT ( 'NONE',  ( -95.43579444196572581, -292.3107578065699954, -220.2753969559761629 ) ) ;
#72264=CARTESIAN_POINT ( 'NONE',  ( 11.36757677955011836, -281.4003875513156459, -215.8514948777255995 ) ) ;
#72265=CARTESIAN_POINT ( 'NONE',  ( -112.2111373206284384, -271.8235697714506500, -253.4086081768912493 ) ) ;
#72266=CARTESIAN_POINT ( 'NONE',  ( -34.66205487393217766, -289.6707164229902673, -347.2124828903785101 ) ) ;
#72267=CARTESIAN_POINT ( 'NONE',  ( -109.0631639589167037, -282.3790468691072419, -294.7811324298340878 ) ) ;
#72268=CARTESIAN_POINT ( 'NONE',  ( 17.78936521832414641, -287.2030237710941947, -222.4794605279162738 ) ) ;
#72270=CARTESIAN_POINT ( 'NONE',  ( -23.57028549459368350, -107.7374504296638662, -360.4863739655157815 ) ) ;
#72271=CARTESIAN_POINT ( 'NONE',  ( 25.36017924250387878, -24.03642681077339915, -341.3531356295546288 ) ) ;
#72272=CARTESIAN_POINT ( 'NONE',  ( -106.5942687000072056, -278.0640325335781995, -246.6114683452737495 ) ) ;
#72273=CARTESIAN_POINT ( 'NONE',  ( 7.341573138019706235, -279.5977177848541260, -212.1794895625533002 ) ) ;
#72274=CARTESIAN_POINT ( 'NONE',  ( 38.47202511600811903, -275.0510172371289173, -256.9432352617927222 ) ) ;
#72275=CARTESIAN_POINT ( 'NONE',  ( -109.2277675425154229, -270.7592608887684946, -295.7727018951397326 ) ) ;
#72276=CARTESIAN_POINT ( 'NONE',  ( -31.10362161087083166, -278.7040981735294736, -194.1531172460235837 ) ) ;
#72277=CARTESIAN_POINT ( 'NONE',  ( -59.45901281187757093, -281.3599024980197782, -341.7083188862335419 ) ) ;
#72278=CARTESIAN_POINT ( 'NONE',  ( -80.07392774482289610, -299.2430099015089695, -207.4652815461180069 ) ) ;
#72279=CARTESIAN_POINT ( 'NONE',  ( -2.415528882757435269, -293.0197865345959372, -206.1740899343403157 ) ) ;
#72280=CARTESIAN_POINT ( 'NONE',  ( 21.55874294835324889, -286.8498353832324028, -314.3364873346901049 ) ) ;
#72281=CARTESIAN_POINT ( 'NONE',  ( -36.94859426095777621, -274.7083943921225568, -193.4510206035448334 ) ) ;
#72282=CARTESIAN_POINT ( 'NONE',  ( -78.85507156741245183, -273.4755238091127580, -210.2527338886961275 ) ) ;
#72285=CARTESIAN_POINT ( 'NONE',  ( -106.1187317843155995, -280.8812939402719167, -238.9455336487226305 ) ) ;
#72286=CARTESIAN_POINT ( 'NONE',  ( 30.30144955051550681, -282.2543290918661683, -242.1010688962793438 ) ) ;
#72287=CARTESIAN_POINT ( 'NONE',  ( -47.99912488591811410, -281.6786475190534134, -195.0723948610824152 ) ) ;
#72288=CARTESIAN_POINT ( 'NONE',  ( -56.39161494658031160, -282.3624832654638794, -341.0753965466946624 ) ) ;
#72290=CARTESIAN_POINT ( 'NONE',  ( -111.3987606656840370, -280.3368417084622592, -276.1992221695654166 ) ) ;
#72291=CARTESIAN_POINT ( 'NONE',  ( -92.52461752139608109, -271.7233265820392489, -221.5189908646295578 ) ) ;
#72294=CARTESIAN_POINT ( 'NONE',  ( 32.40218928169948498, -275.9400971503192181, -237.9862127939964012 ) ) ;
#72296=CARTESIAN_POINT ( 'NONE',  ( 19.32627761765927232, -278.2340522669654206, -319.5104013540642427 ) ) ;
#72297=CARTESIAN_POINT ( 'NONE',  ( -17.52831131349818605, -275.3761079486423000, -344.1583802288861307 ) ) ;
#72300=CARTESIAN_POINT ( 'NONE',  ( -60.69740747673365178, -285.3334311645833736, -342.0599896476688855 ) ) ;
#72301=CARTESIAN_POINT ( 'NONE',  ( 4.604573070467113283, -291.8313952696607885, -210.3564378658357725 ) ) ;
#72302=CARTESIAN_POINT ( 'NONE',  ( -60.47134776451586191, -285.1085826269522272, -196.9685044823650060 ) ) ;
#72304=CARTESIAN_POINT ( 'NONE',  ( -111.3215431993391888, -282.8209711353330817, -268.1347240019587161 ) ) ;
#72305=CARTESIAN_POINT ( 'NONE',  ( -92.11566487178816942, -282.4290034838576844, -319.5246440141611970 ) ) ;
#72306=CARTESIAN_POINT ( 'NONE',  ( 35.99018845063282157, -285.4626873220703374, -257.2733993661242948 ) ) ;
#72307=CARTESIAN_POINT ( 'NONE',  ( -21.28649211525090479, -284.0468304549337972, -342.0329719214699367 ) ) ;
#72308=CARTESIAN_POINT ( 'NONE',  ( 14.65917142435139020, -272.7842003548737466, -216.3156740968620682 ) ) ;
#72309=CARTESIAN_POINT ( 'NONE',  ( -113.5406754944499994, -282.9570249480919983, -269.9654331216248124 ) ) ;
#72310=CARTESIAN_POINT ( 'NONE',  ( -80.69432203633989786, -297.6399208043936255, -331.6254403074904076 ) ) ;
#72311=CARTESIAN_POINT ( 'NONE',  ( -1.813072759501491493, -284.5216069130643746, -204.1210616263202269 ) ) ;
#72312=CARTESIAN_POINT ( 'NONE',  ( -107.3379690782405049, -279.2069978524250473, -292.0698910013197178 ) ) ;
#72313=CARTESIAN_POINT ( 'NONE',  ( 35.37740486799152251, -289.7962630883467341, -289.3863695722653802 ) ) ;
#72316=CARTESIAN_POINT ( 'NONE',  ( 8.060766910421152787, -296.3569860463745158, -330.7592154862559823 ) ) ;
#72317=CARTESIAN_POINT ( 'NONE',  ( -110.4411794156051343, -276.3358494383647326, -287.1950874932304600 ) ) ;
#72318=CARTESIAN_POINT ( 'NONE',  ( -98.03835466682205890, -289.1187727297029824, -317.4787892858459486 ) ) ;
#72319=CARTESIAN_POINT ( 'NONE',  ( -23.38732462683824309, -293.2707813432017474, -342.8820085607288206 ) ) ;
#72320=CARTESIAN_POINT ( 'NONE',  ( -32.91669927876350954, -278.7938902948168334, -197.0013003295241276 ) ) ;
#72321=CARTESIAN_POINT ( 'NONE',  ( -73.42692764383861004, -295.7076050945018437, -205.4864554666810932 ) ) ;
#72322=CARTESIAN_POINT ( 'NONE',  ( -60.42967334378176503, -293.0616995951370427, -200.5353064467257695 ) ) ;
#72323=CARTESIAN_POINT ( 'NONE',  ( -95.99890600148557951, -281.6948066931273615, -223.6242672951989618 ) ) ;
#72324=CARTESIAN_POINT ( 'NONE',  ( 21.73743018943032368, -292.6864266111173265, -318.6761792991862876 ) ) ;
#72325=CARTESIAN_POINT ( 'NONE',  ( -83.02569930113418195, -291.2896577480779001, -328.3215582203089298 ) ) ;
#72326=CARTESIAN_POINT ( 'NONE',  ( -103.7138287943378714, -289.2780502935710842, -233.3649756436069538 ) ) ;
#72328=CARTESIAN_POINT ( 'NONE',  ( 31.96035507837568446, -289.3043318698337885, -295.1118767721363270 ) ) ;
#72330=CARTESIAN_POINT ( 'NONE',  ( -86.83110237122282626, -290.5643688097696895, -324.3130494404123283 ) ) ;
#72332=CIRCLE ( 'NONE', #48101, 5.841085083515828558 ) ;
#72333=CARTESIAN_POINT ( 'NONE',  ( -17.81068312611191118, -290.0107717184785088, -344.4323545887829141 ) ) ;
#72334=CARTESIAN_POINT ( 'NONE',  ( -38.12692121901730502, -278.0624698668577253, -195.0100049518649143 ) ) ;
#72335=CARTESIAN_POINT ( 'NONE',  ( -101.8758126719622936, -279.4378021132837375, -228.2992820170711923 ) ) ;
#72336=CARTESIAN_POINT ( 'NONE',  ( 37.17027205420120595, -281.4608930582771791, -289.6927059440723724 ) ) ;
#72337=CARTESIAN_POINT ( 'NONE',  ( 25.91180322605778130, -286.0943649804596589, -310.6599388254431346 ) ) ;
#72339=CARTESIAN_POINT ( 'NONE',  ( -1.858755135424154492, -280.7165115041714216, -335.5816749656914340 ) ) ;
#72340=CARTESIAN_POINT ( 'NONE',  ( -110.2802654800144637, -282.3270707908436634, -287.8788439460030304 ) ) ;
#72341=CARTESIAN_POINT ( 'NONE',  ( 202.9738562182569694, 291.9636489450776367, -53.99999999998589573 ) ) ;
#72342=CARTESIAN_POINT ( 'NONE',  ( -98.01320858352929122, -277.6548301704020787, -224.0615960724933871 ) ) ;
#72344=CARTESIAN_POINT ( 'NONE',  ( -87.53719931808655019, -284.2913338563616321, -212.3088931166980160 ) ) ;
#72345=CARTESIAN_POINT ( 'NONE',  ( -41.89490681170891406, -298.9346230229483581, -197.2675015902693474 ) ) ;
#72346=CARTESIAN_POINT ( 'NONE',  ( -103.1318838608503370, -292.6028230561269083, -236.8100478987950055 ) ) ;
#72347=CARTESIAN_POINT ( 'NONE',  ( 39.03532149031855880, -277.0232541309891303, -273.9976813426529816 ) ) ;
#72348=CARTESIAN_POINT ( 'NONE',  ( 35.04202796950075083, -275.0919070058828879, -260.7338965005125715 ) ) ;
#72349=CARTESIAN_POINT ( 'NONE',  ( -48.05419328290528114, -297.1884613256227681, -344.6448126325227008 ) ) ;
#72350=CARTESIAN_POINT ( 'NONE',  ( 12.41744354550193030, -288.5476419365103879, -329.1235858115808810 ) ) ;
#72352=CARTESIAN_POINT ( 'NONE',  ( 35.22376406062967646, -279.3623275507391668, -249.2536355017128642 ) ) ;
#72353=CARTESIAN_POINT ( 'NONE',  ( -47.74129086144256462, -291.7568585391829856, -194.0128379952026876 ) ) ;
#72354=CARTESIAN_POINT ( 'NONE',  ( -49.71672652828929984, -290.9493209418427568, -198.1274475385925768 ) ) ;
#72355=CARTESIAN_POINT ( 'NONE',  ( 7.684596219073196011, -292.4373024779761749, -330.3413920984033325 ) ) ;
#72358=CARTESIAN_POINT ( 'NONE',  ( -89.85619900138516414, -290.7932219936263323, -219.5652928614318000 ) ) ;
#72360=CARTESIAN_POINT ( 'NONE',  ( -60.45054442856106647, -286.7009913387566939, -197.1018731090796337 ) ) ;
#72361=CARTESIAN_POINT ( 'NONE',  ( 30.89617123739170168, -273.2666405000204009, -285.9686137636504668 ) ) ;
#72362=CARTESIAN_POINT ( 'NONE',  ( -34.87424860828389939, -294.0806163091604049, -347.0861588532150677 ) ) ;
#72363=CARTESIAN_POINT ( 'NONE',  ( -111.2492318530325690, -286.1187586573374233, -250.3887463344401851 ) ) ;
#72364=CARTESIAN_POINT ( 'NONE',  ( -77.04728420643806430, -285.3374312969164066, -209.0437629944918854 ) ) ;
#72365=CARTESIAN_POINT ( 'NONE',  ( 30.80869125610385950, -276.6984068812309943, -242.1873839013264558 ) ) ;
#72366=CARTESIAN_POINT ( 'NONE',  ( -6.098930381301286729, -292.6596313054743064, -338.1529769696238645 ) ) ;
#72367=CARTESIAN_POINT ( 'NONE',  ( 35.32346731477522894, -295.4952606656176499, -284.4233886388359451 ) ) ;
#72368=CARTESIAN_POINT ( 'NONE',  ( -24.27390023893061155, -275.6766422279484345, -342.6372412801852647 ) ) ;
#72371=CARTESIAN_POINT ( 'NONE',  ( -56.06924778861748138, -294.9537140593471349, -345.0271962916477264 ) ) ;
#72372=CARTESIAN_POINT ( 'NONE',  ( 34.04407598824657555, -289.1979204152081593, -249.2120527142809010 ) ) ;
#72373=CARTESIAN_POINT ( 'NONE',  ( -37.76724320851720051, -296.0466686025325771, -195.3609641834697754 ) ) ;
#72374=CARTESIAN_POINT ( 'NONE',  ( -70.60744661030534530, -298.7033710379445210, -201.2605924963585835 ) ) ;
#72375=CARTESIAN_POINT ( 'NONE',  ( 4.777335013650172435, -287.2889754373408095, -210.5507093577442674 ) ) ;
#72377=CARTESIAN_POINT ( 'NONE',  ( -100.0498363963993285, -278.1986015786310986, -226.0834728447778730 ) ) ;
#72378=CARTESIAN_POINT ( 'NONE',  ( 32.14148067564948263, -294.6277154756776895, -303.4306896044388395 ) ) ;
#72379=CARTESIAN_POINT ( 'NONE',  ( -8.722035735439540360, -286.8212591130728129, -340.5265630167794484 ) ) ;
#72380=CARTESIAN_POINT ( 'NONE',  ( -39.10310031736396752, -295.4069700298720704, -347.3198196412745915 ) ) ;
#72381=CARTESIAN_POINT ( 'NONE',  ( -14.84391723107736638, -292.6851178169182504, -200.8921518794097949 ) ) ;
#72384=CARTESIAN_POINT ( 'NONE',  ( -110.6395504404451202, -271.5021484970271217, -270.3477489206637756 ) ) ;
#72385=CARTESIAN_POINT ( 'NONE',  ( 15.80231778419920197, -288.3086272243522785, -215.6032773406455760 ) ) ;
#72386=CARTESIAN_POINT ( 'NONE',  ( -55.63300648810263738, -292.7666405000204577, -350.3538533559490702 ) ) ;
#72388=CARTESIAN_POINT ( 'NONE',  ( -108.4152802970828589, -278.2743668322917188, -241.0036830082741233 ) ) ;
#72389=CARTESIAN_POINT ( 'NONE',  ( -62.11828371793386339, -285.3750885773587811, -341.0283543836637250 ) ) ;
#72390=CARTESIAN_POINT ( 'NONE',  ( -75.79438099187554201, -284.1244679167076583, -204.2699171581229507 ) ) ;
#72391=CARTESIAN_POINT ( 'NONE',  ( 13.11422935688720237, -286.4208306744771448, -325.1624225558999228 ) ) ;
#72392=CARTESIAN_POINT ( 'NONE',  ( 21.69369989309521074, -278.0595462401945497, -317.8698256562278175 ) ) ;
#72393=CARTESIAN_POINT ( 'NONE',  ( -47.28732485252812978, -298.4148558079792792, -197.9284228179813283 ) ) ;
#72395=CARTESIAN_POINT ( 'NONE',  ( 34.54647888706180225, -292.4379195302273615, -285.6966662491015541 ) ) ;
#72396=CARTESIAN_POINT ( 'NONE',  ( -96.09300449106507358, -277.9446425157504450, -313.7097088486643770 ) ) ;
#72397=CARTESIAN_POINT ( 'NONE',  ( -49.15021637553330436, -279.2462641699862047, -198.2192327012321016 ) ) ;
#72398=CARTESIAN_POINT ( 'NONE',  ( 7.044840683782811475, -275.7202922558966520, -207.7553474174759742 ) ) ;
#72399=CARTESIAN_POINT ( 'NONE',  ( -71.44579397653382102, -276.4123722067806170, -339.0517526711394112 ) ) ;
#72400=CARTESIAN_POINT ( 'NONE',  ( 151.8322611248232761, 206.3920080503552299, -215.3183130715498237 ) ) ;
#72401=EDGE_CURVE ( 'NONE', #3540, #29794, #66598, .T. ) ;
#72402=CARTESIAN_POINT ( 'NONE',  ( -93.24590105861459222, -297.2616604054534264, -322.4699851835310938 ) ) ;
#72404=EDGE_LOOP ( 'NONE', ( #48714, #33937, #91193, #74675 ) ) ;
#72406=CARTESIAN_POINT ( 'NONE',  ( 82.62533370646633557, -301.4052215159320554, -193.6716506432818505 ) ) ;
#72407=CARTESIAN_POINT ( 'NONE',  ( -73.72092288612660127, -286.6367395514758414, -206.7008348303947116 ) ) ;
#72408=CARTESIAN_POINT ( 'NONE',  ( -30.99117931021702077, -287.8914667457218002, -194.6271629235722003 ) ) ;
#72409=CARTESIAN_POINT ( 'NONE',  ( 8.036741488494483221, -287.7612405829243585, -327.6733305055087726 ) ) ;
#72410=CARTESIAN_POINT ( 'NONE',  ( -0.4104896363085420719, -282.0823907548179363, -337.8713228869076488 ) ) ;
#72411=CARTESIAN_POINT ( 'NONE',  ( -104.0847441641706723, -277.3743710621465084, -238.7481140434367433 ) ) ;
#72412=CARTESIAN_POINT ( 'NONE',  ( -111.3248661378664366, -286.3332882958701475, -276.4731246619610943 ) ) ;
#72413=CARTESIAN_POINT ( 'NONE',  ( -72.44307058668638888, -278.0584812247415698, -205.5645012077888509 ) ) ;
#72414=CARTESIAN_POINT ( 'NONE',  ( -78.89714023838975265, -278.9401774919166996, -331.0398147248430973 ) ) ;
#72415=CARTESIAN_POINT ( 'NONE',  ( 35.43892178647172386, -275.9528650136715555, -263.4086585093682515 ) ) ;
#72416=CARTESIAN_POINT ( 'NONE',  ( 22.96531292912590416, -286.9819393652680901, -317.6164683223841507 ) ) ;
#72417=CARTESIAN_POINT ( 'NONE',  ( -4.224152200932622669, -283.4294509516602147, -339.7108995702823222 ) ) ;
#72418=CARTESIAN_POINT ( 'NONE',  ( -13.43510110557483195, -283.2421690279384165, -343.4911489294484568 ) ) ;
#72422=CARTESIAN_POINT ( 'NONE',  ( -45.86293297917267608, -291.0193708864263726, -345.6974809327636535 ) ) ;
#72423=CARTESIAN_POINT ( 'NONE',  ( -96.91669144151408943, -288.5891781684961188, -318.3830196501817227 ) ) ;
#72424=CARTESIAN_POINT ( 'NONE',  ( -54.25427897830437729, -272.8882896585868139, -199.1054296201107547 ) ) ;
#72425=CARTESIAN_POINT ( 'NONE',  ( 27.97017481252142446, -292.3679205973182889, -229.6689625656405838 ) ) ;
#72426=CARTESIAN_POINT ( 'NONE',  ( -42.73378834055788644, -287.6011457977434702, -343.9080062660941053 ) ) ;
#72427=CARTESIAN_POINT ( 'NONE',  ( -0.7362689309894312473, -290.7852711599860527, -206.0190237905486583 ) ) ;
#72428=CARTESIAN_POINT ( 'NONE',  ( 30.85981004913265124, -289.1198039435548708, -297.6217723295335986 ) ) ;
#72429=CARTESIAN_POINT ( 'NONE',  ( -20.25526795762937127, -294.7662352645559167, -195.3538533559490702 ) ) ;
#72430=CARTESIAN_POINT ( 'NONE',  ( 6.779081402897817021, -290.4525920728215738, -331.0746385504962745 ) ) ;
#72431=CARTESIAN_POINT ( 'NONE',  ( -66.28539371404242786, -289.6739569138085244, -200.9904395240850761 ) ) ;
#72432=CARTESIAN_POINT ( 'NONE',  ( -112.3718944099562691, -292.5751568835734133, -268.5823054727151202 ) ) ;
#72433=CARTESIAN_POINT ( 'NONE',  ( -110.2298382067374689, -285.5936551189691386, -262.7374332444052243 ) ) ;
#72434=CARTESIAN_POINT ( 'NONE',  ( 23.31948440883498108, -294.9485837904136929, -225.9736296617211906 ) ) ;
#72436=CARTESIAN_POINT ( 'NONE',  ( -91.01558547671376687, -275.2743451916153390, -217.4695228705287775 ) ) ;
#72437=CARTESIAN_POINT ( 'NONE',  ( 34.49474068519236170, -280.5660015079667460, -256.4340652475358411 ) ) ;
#72438=CARTESIAN_POINT ( 'NONE',  ( -26.47756707605085680, -280.9138818161818563, -344.6227910774465499 ) ) ;
#72439=CARTESIAN_POINT ( 'NONE',  ( -47.62011244711185043, -294.3768334893219958, -346.5090861784170784 ) ) ;
#72440=CARTESIAN_POINT ( 'NONE',  ( -27.12847242738258302, -272.4234578560213436, -197.0042323288284933 ) ) ;
#72441=CARTESIAN_POINT ( 'NONE',  ( -107.6318756588853347, -276.3104907502766423, -295.0248476005363045 ) ) ;
#72442=CARTESIAN_POINT ( 'NONE',  ( -92.22424347755826091, -298.5615567458141868, -221.4821867932911630 ) ) ;
#72443=CARTESIAN_POINT ( 'NONE',  ( -6.501571968834195303, -296.0642447797637828, -337.1762466134138663 ) ) ;
#72444=LINE ( 'NONE', #65363, #36905 ) ;
#72445=CARTESIAN_POINT ( 'NONE',  ( 20.65745723903233255, -294.9814197655427392, -314.9764700530721484 ) ) ;
#72447=CARTESIAN_POINT ( 'NONE',  ( 35.54690944578270972, -285.8168539298790733, -289.4832883625795716 ) ) ;
#72448=CARTESIAN_POINT ( 'NONE',  ( -91.84489242409644305, -297.2465951656284915, -221.7977364122492645 ) ) ;
#72449=CARTESIAN_POINT ( 'NONE',  ( -114.2083498269823281, -284.4851597106874692, -275.7177805342258807 ) ) ;
#72450=CARTESIAN_POINT ( 'NONE',  ( 38.76531059052156536, -287.0732505586276488, -258.7205217537386375 ) ) ;
#72451=CARTESIAN_POINT ( 'NONE',  ( -3.993769976123546783, -290.4927471217835091, -203.3547228439092009 ) ) ;
#72452=CARTESIAN_POINT ( 'NONE',  ( -40.99047764218310874, -279.2045355661306871, -193.5961081341890235 ) ) ;
#72453=CARTESIAN_POINT ( 'NONE',  ( -4.771743288812454686, -277.9809262143061233, -202.8022627189028810 ) ) ;
#72455=CARTESIAN_POINT ( 'NONE',  ( 33.41612651763995245, -286.0907303174925573, -250.8557219609286904 ) ) ;
#72457=CARTESIAN_POINT ( 'NONE',  ( -98.78974503100785398, -288.8593147845825797, -316.2699865052107953 ) ) ;
#72458=CARTESIAN_POINT ( 'NONE',  ( 129.4467878515196162, -299.5541904835127980, -195.3611179825600175 ) ) ;
#72459=CARTESIAN_POINT ( 'NONE',  ( -97.82749601706665032, -297.5690545741524033, -312.6447899086027178 ) ) ;
#72460=CARTESIAN_POINT ( 'NONE',  ( -35.36956734517416123, -281.5016849120055440, -193.9627623263442047 ) ) ;
#72461=CARTESIAN_POINT ( 'NONE',  ( -111.2700146654799198, -294.7596233637084424, -255.6999702150303904 ) ) ;
#72462=CARTESIAN_POINT ( 'NONE',  ( 23.70253940223141953, -280.6623913137541422, -230.1988833781170172 ) ) ;
#72463=CARTESIAN_POINT ( 'NONE',  ( -16.50483899443910474, -294.9569303705647485, -344.5434395678910278 ) ) ;
#72464=CARTESIAN_POINT ( 'NONE',  ( 25.94527036239873752, -285.0793805991111185, -229.0806920683648400 ) ) ;
#72466=CARTESIAN_POINT ( 'NONE',  ( -78.82630241131643345, -281.4937130287340210, -207.8165809848790389 ) ) ;
#72468=CARTESIAN_POINT ( 'NONE',  ( -107.0970534282177908, -295.3140784668618721, -292.8323044787042591 ) ) ;
#72470=PLANE ( 'NONE',  #60497 ) ;
#72471=CARTESIAN_POINT ( 'NONE',  ( -70.93302701220437712, -285.4774176831608656, -337.0347642082821267 ) ) ;
#72473=CARTESIAN_POINT ( 'NONE',  ( -4.829096099716524648, -292.1237833571632905, -337.9475929042657754 ) ) ;
#72474=CARTESIAN_POINT ( 'NONE',  ( -7.743308129422456609, -273.6273474602290321, -199.3955810154421613 ) ) ;
#72475=CARTESIAN_POINT ( 'NONE',  ( -98.29836869864304560, -290.9436200617894315, -230.1035884041222914 ) ) ;
#72476=CARTESIAN_POINT ( 'NONE',  ( 33.99955040372994830, -283.3144039726696519, -288.8812401604149613 ) ) ;
#72477=CARTESIAN_POINT ( 'NONE',  ( -34.02489317914503175, -275.6946953407403385, -196.6356867657671330 ) ) ;
#72478=CARTESIAN_POINT ( 'NONE',  ( 29.07472106646553911, -283.6432110681266749, -307.8224134474925791 ) ) ;
#72479=CARTESIAN_POINT ( 'NONE',  ( -1.069050037832547373, -281.3541058323182256, -334.1688397771936252 ) ) ;
#72480=CARTESIAN_POINT ( 'NONE',  ( -111.4649080150244771, -280.4054939245332889, -281.7957453037777782 ) ) ;
#72481=CARTESIAN_POINT ( 'NONE',  ( -35.82814869556214887, -298.0706118946271772, -193.3611179679607517 ) ) ;
#72482=CARTESIAN_POINT ( 'NONE',  ( -38.35528272054697396, -273.8730960703282449, -193.3677893438971012 ) ) ;
#72483=CARTESIAN_POINT ( 'NONE',  ( 35.89559336655222666, -295.2989859739282679, -256.9632095782571355 ) ) ;
#72486=CARTESIAN_POINT ( 'NONE',  ( 25.47419231884276769, -292.2589954653012114, -312.7222928556045645 ) ) ;
#72487=CARTESIAN_POINT ( 'NONE',  ( 9.529357840163710236, -274.2245411284644661, -214.2494125576347130 ) ) ;
#72488=CARTESIAN_POINT ( 'NONE',  ( -69.35014769092640563, -293.1587404554376235, -201.0781015635876372 ) ) ;
#72489=CARTESIAN_POINT ( 'NONE',  ( -69.91165696735023971, -276.1233781216988064, -202.8022627189028810 ) ) ;
#72490=CARTESIAN_POINT ( 'NONE',  ( -50.51324527192370795, -293.0926039505428662, -194.8990804000737569 ) ) ;
#72491=CARTESIAN_POINT ( 'NONE',  ( 6.949720710678732871, -290.4483194737858867, -330.7440225901233930 ) ) ;
#72492=CARTESIAN_POINT ( 'NONE',  ( -74.95628212740679430, -275.5542320899593278, -335.0540205912255374 ) ) ;
#72493=CARTESIAN_POINT ( 'NONE',  ( -98.82466471295813903, -279.8997062925695900, -312.3272860733979996 ) ) ;
#72494=CARTESIAN_POINT ( 'NONE',  ( 32.18184845277908579, -291.2835686890792886, -243.7567877200997373 ) ) ;
#72495=CARTESIAN_POINT ( 'NONE',  ( 20.67961527332043659, -284.0792396965493367, -319.0831093466072730 ) ) ;
#72497=CARTESIAN_POINT ( 'NONE',  ( -92.57790451437017509, -283.5383840610160746, -318.1404784485881123 ) ) ;
#72498=CARTESIAN_POINT ( 'NONE',  ( -3.805246342170619744, -281.5639037684901496, -201.3771099570574847 ) ) ;
#72499=CARTESIAN_POINT ( 'NONE',  ( -90.17544299733241076, -282.5738928029912813, -325.9010110979442629 ) ) ;
#72500=CARTESIAN_POINT ( 'NONE',  ( -84.43207734220997907, -280.3633900977930011, -209.6694526033395789 ) ) ;
#72502=CARTESIAN_POINT ( 'NONE',  ( 37.23225998466632092, -277.2770902609273094, -286.5911028344676197 ) ) ;
#72503=CARTESIAN_POINT ( 'NONE',  ( -102.0172624299486870, -292.6233781216987495, -301.5434626090942061 ) ) ;
#72505=CARTESIAN_POINT ( 'NONE',  ( -71.39786857046402702, -299.6026364355964233, -203.5248355771068987 ) ) ;
#72506=CARTESIAN_POINT ( 'NONE',  ( -112.0379594211455299, -276.5689253040086442, -270.6191293348912268 ) ) ;
#72507=CARTESIAN_POINT ( 'NONE',  ( -109.4761318875154927, -292.6188475049196995, -246.3091178506803374 ) ) ;
#72508=CARTESIAN_POINT ( 'NONE',  ( 34.42286396606191090, -293.0840961461039456, -284.2801699919195926 ) ) ;
#72509=CARTESIAN_POINT ( 'NONE',  ( -74.40318166068551875, -289.0390548109408542, -337.7999947942155359 ) ) ;
#72511=CARTESIAN_POINT ( 'NONE',  ( 39.12199617771334204, -292.1264693963765922, -270.3284663171629063 ) ) ;
#72512=CARTESIAN_POINT ( 'NONE',  ( -104.2016957520456657, -283.3707929919136177, -238.9961436908962753 ) ) ;
#72513=CARTESIAN_POINT ( 'NONE',  ( -103.9433589941564975, -291.9756494575484567, -303.1495994008913044 ) ) ;
#72514=CARTESIAN_POINT ( 'NONE',  ( -37.26085850520976805, -284.5330222512640148, -196.6552701262254175 ) ) ;
#72515=CARTESIAN_POINT ( 'NONE',  ( 8.112016673473407380, -283.7311679443093908, -328.1773409008856106 ) ) ;
#72516=CARTESIAN_POINT ( 'NONE',  ( -110.5538003603362540, -291.2004684704143074, -293.6173345970029231 ) ) ;
#72517=CARTESIAN_POINT ( 'NONE',  ( -54.51332980933040062, -280.3179963928682241, -199.2939224595110375 ) ) ;
#72518=CARTESIAN_POINT ( 'NONE',  ( 37.37742595089603981, -292.1341660051416511, -253.4185054195157250 ) ) ;
#72519=CARTESIAN_POINT ( 'NONE',  ( 20.45819815466221669, -289.0415479219254280, -321.0102881602378488 ) ) ;
#72520=CARTESIAN_POINT ( 'NONE',  ( 37.31559320140213032, -287.8116573555047921, -251.7650039744999049 ) ) ;
#72521=CARTESIAN_POINT ( 'NONE',  ( -77.05084475036461811, -285.6707376738506809, -209.0460689899842350 ) ) ;
#72524=CARTESIAN_POINT ( 'NONE',  ( -19.55391271551662413, -296.6863134951481129, -344.0622593021132047 ) ) ;
#72525=CARTESIAN_POINT ( 'NONE',  ( -110.7469981448205090, -294.9642398368066551, -291.9703047470334241 ) ) ;
#72526=CARTESIAN_POINT ( 'NONE',  ( -107.3450741805652484, -277.3247976227939944, -292.0469738322642002 ) ) ;
#72527=CARTESIAN_POINT ( 'NONE',  ( 30.68463594159268837, -298.2314732075915913, -193.4703145117252063 ) ) ;
#72529=CARTESIAN_POINT ( 'NONE',  ( -97.76283247898805939, -294.4493080345956741, -312.5510992403744694 ) ) ;
#72530=CARTESIAN_POINT ( 'NONE',  ( 27.66738970187153868, -277.7898860117940103, -305.8489921116553774 ) ) ;
#72531=CARTESIAN_POINT ( 'NONE',  ( -100.3159900907502760, -271.2252678196702504, -231.0533034547927116 ) ) ;
#72532=CARTESIAN_POINT ( 'NONE',  ( 0.09847226857732659100, -293.7677214703746245, -207.2313785898181209 ) ) ;
#72533=CARTESIAN_POINT ( 'NONE',  ( -28.84656577089856100, -296.0217406351200111, -343.2275856026936935 ) ) ;
#72535=CARTESIAN_POINT ( 'NONE',  ( -95.99330775262825455, -293.9065832461334935, -317.3923178194326056 ) ) ;
#72536=CARTESIAN_POINT ( 'NONE',  ( -73.24043553275097906, -298.2406541149025543, -202.2979816630649168 ) ) ;
#72537=CARTESIAN_POINT ( 'NONE',  ( -92.61322325112715248, -275.2606048656767825, -219.6463460953772824 ) ) ;
#72538=CARTESIAN_POINT ( 'NONE',  ( -110.2081949564013570, -291.5899308944818245, -263.0206561951536628 ) ) ;
#72539=CARTESIAN_POINT ( 'NONE',  ( -61.01600955640119395, -295.7012379566804157, -339.4915810968141159 ) ) ;
#72540=CARTESIAN_POINT ( 'NONE',  ( -111.3848459749370647, -280.7118448247438778, -256.2912972431313960 ) ) ;
#72541=CARTESIAN_POINT ( 'NONE',  ( -81.93773299491124362, -278.1431198513420782, -208.1960785785962003 ) ) ;
#72542=CARTESIAN_POINT ( 'NONE',  ( 0.8105687729348383108, -281.9057659049092877, -337.1424670130624008 ) ) ;
#72543=CARTESIAN_POINT ( 'NONE',  ( 22.55637436049275735, -275.5481237413729332, -318.6057283681213335 ) ) ;
#72544=CARTESIAN_POINT ( 'NONE',  ( -108.7806349874023368, -282.3600037446211104, -291.3301799447464759 ) ) ;
#72545=CARTESIAN_POINT ( 'NONE',  ( -105.4512804616232557, -277.3975232945321068, -236.0745903104890999 ) ) ;
#72546=CARTESIAN_POINT ( 'NONE',  ( -20.15017322816388301, -278.2722409075090582, -197.1333356819495179 ) ) ;
#72547=CARTESIAN_POINT ( 'NONE',  ( -106.8570959947575858, -271.4454226281304727, -246.2160428287999139 ) ) ;
#72548=CARTESIAN_POINT ( 'NONE',  ( 37.45331456715422291, -277.4727434856657169, -264.1638155495293745 ) ) ;
#72550=CARTESIAN_POINT ( 'NONE',  ( 26.66880200969132275, -291.0396556977514138, -230.4998943694332638 ) ) ;
#72551=CARTESIAN_POINT ( 'NONE',  ( -110.7818462594062794, -290.2593683143845169, -293.6771520792515275 ) ) ;
#72552=CARTESIAN_POINT ( 'NONE',  ( 34.81848707872747184, -277.2798301914128274, -249.1334051030851526 ) ) ;
#72553=CARTESIAN_POINT ( 'NONE',  ( -55.71986598453124628, -295.8150078339552920, -197.7659835107414494 ) ) ;
#72554=CARTESIAN_POINT ( 'NONE',  ( -114.0478625993830946, -283.6824563952880567, -275.6963609930496091 ) ) ;
#72556=CARTESIAN_POINT ( 'NONE',  ( -94.89748846829182582, -281.8875155036677711, -318.4673863696773424 ) ) ;
#72558=CARTESIAN_POINT ( 'NONE',  ( -4.642465675522531754, -291.2877032153002119, -204.6364584404161917 ) ) ;
#72559=CARTESIAN_POINT ( 'NONE',  ( -110.6369739595502750, -282.8455323536790615, -258.5050059402002489 ) ) ;
#72562=CARTESIAN_POINT ( 'NONE',  ( -33.37794337555711621, -290.1018730301097435, -195.4530950868605430 ) ) ;
#72563=CARTESIAN_POINT ( 'NONE',  ( -112.3133133919373137, -283.2148036820084940, -255.8751328056139585 ) ) ;
#72564=CARTESIAN_POINT ( 'NONE',  ( -9.669690345268849185, -278.2846611672024437, -338.7904777536710412 ) ) ;
#72565=CARTESIAN_POINT ( 'NONE',  ( -106.6398797693199754, -285.3368789335958695, -303.0072665436413217 ) ) ;
#72566=CARTESIAN_POINT ( 'NONE',  ( -94.12204122672858375, -285.2012035854315855, -224.4611050949243349 ) ) ;
#72567=CARTESIAN_POINT ( 'NONE',  ( -96.55642434655884188, -279.3696844236321226, -314.0742388105763325 ) ) ;
#72568=CARTESIAN_POINT ( 'NONE',  ( -108.9206426547602007, -279.1557767770505620, -285.4957377086757333 ) ) ;
#72569=EDGE_CURVE ( 'NONE', #54554, #55239, #15659, .T. ) ;
#72570=CARTESIAN_POINT ( 'NONE',  ( -106.3759907889436676, -286.1676952669240563, -299.8071333148836288 ) ) ;
#72572=CARTESIAN_POINT ( 'NONE',  ( -112.3062886209723246, -296.1648073402035948, -288.0053794569739125 ) ) ;
#72573=CARTESIAN_POINT ( 'NONE',  ( 37.09415822743715552, -289.6124613335972526, -276.5941347606562317 ) ) ;
#72575=CARTESIAN_POINT ( 'NONE',  ( 40.64545035920995986, -277.8376638359844719, -252.5284128619064461 ) ) ;
#72577=CARTESIAN_POINT ( 'NONE',  ( 22.53031338191065558, -292.5892404096684913, -317.5178330610325474 ) ) ;
#72578=CARTESIAN_POINT ( 'NONE',  ( -7.996478995075433360, -287.9638556434179577, -202.7625547549774865 ) ) ;
#72579=CARTESIAN_POINT ( 'NONE',  ( -43.86239788051945254, -281.7288987808649949, -196.5846516963759143 ) ) ;
#72580=CARTESIAN_POINT ( 'NONE',  ( 37.14116041450215988, -288.7618041610055570, -253.2470326521925585 ) ) ;
#72581=CARTESIAN_POINT ( 'NONE',  ( 34.61440998920159018, -289.1994401457372419, -296.5079724830959549 ) ) ;
#72582=CARTESIAN_POINT ( 'NONE',  ( -71.09274929014462430, -285.4976827031066478, -337.3520953439282266 ) ) ;
#72583=CARTESIAN_POINT ( 'NONE',  ( -113.2988186932705190, -278.5608762988898661, -282.9910880453745676 ) ) ;
#72585=CARTESIAN_POINT ( 'NONE',  ( -65.09772464383418367, -293.4918151325490498, -340.6525070171761627 ) ) ;
#72586=CARTESIAN_POINT ( 'NONE',  ( 15.16288599107901547, -280.6019615119516857, -213.9653338154396920 ) ) ;
#72587=CARTESIAN_POINT ( 'NONE',  ( -57.21469351174712159, -275.6535765551521422, -198.7817778015042620 ) ) ;
#72589=CARTESIAN_POINT ( 'NONE',  ( 35.77081079830085031, -289.8376638359844719, -253.6410175316879361 ) ) ;
#72591=CARTESIAN_POINT ( 'NONE',  ( -89.45142107969505219, -271.5703952154502190, -214.9851168817320684 ) ) ;
#72593=CARTESIAN_POINT ( 'NONE',  ( -104.4961695712554359, -278.4460939744859616, -241.5815127857250673 ) ) ;
#72594=CARTESIAN_POINT ( 'NONE',  ( 37.20900640974227258, -276.9792854272424734, -288.0301875914694847 ) ) ;
#72595=AXIS2_PLACEMENT_3D ( 'NONE', #92284, #36407, #42616 ) ;
#72596=CARTESIAN_POINT ( 'NONE',  ( -90.48384561372591861, -298.7067987250415513, -219.3834844801939710 ) ) ;
#72597=CARTESIAN_POINT ( 'NONE',  ( -38.74031533311053010, -282.1280457637220138, -347.1130827091283209 ) ) ;
#72598=CARTESIAN_POINT ( 'NONE',  ( -97.36749464010824795, -291.7150028987358041, -313.6609795076416844 ) ) ;
#72599=CARTESIAN_POINT ( 'NONE',  ( -36.92126781798521762, -299.5774404508446764, -194.0543399737223638 ) ) ;
#72600=CARTESIAN_POINT ( 'NONE',  ( -48.92517658921273238, -299.1129439867789870, -194.5856578921626863 ) ) ;
#72601=CARTESIAN_POINT ( 'NONE',  ( 20.26019253863147185, -296.2132047912186863, -318.1319290640575446 ) ) ;
#72602=CARTESIAN_POINT ( 'NONE',  ( -92.09992261821246018, -281.8365326748772191, -321.3666617661593818 ) ) ;
#72603=CARTESIAN_POINT ( 'NONE',  ( -96.55988284443661485, -290.8806004919076713, -221.1579155437943314 ) ) ;
#72604=CARTESIAN_POINT ( 'NONE',  ( -94.14951462356270895, -271.2460666162605207, -221.9190971143331126 ) ) ;
#72605=CARTESIAN_POINT ( 'NONE',  ( -62.95194199385857559, -287.3242735564728605, -198.5937442934177852 ) ) ;
#72606=CARTESIAN_POINT ( 'NONE',  ( -96.81741606163974723, -288.8756490969257129, -313.2197844149259254 ) ) ;
#72607=CARTESIAN_POINT ( 'NONE',  ( -76.51609685821101436, -209.3017665391693072, -356.9869174788681789 ) ) ;
#72609=CARTESIAN_POINT ( 'NONE',  ( -89.10574573416242572, -288.3381346490827468, -326.5668994832099656 ) ) ;
#72610=CARTESIAN_POINT ( 'NONE',  ( -3.360313273740507700, -288.2575124139892182, -335.0495605402925889 ) ) ;
#72612=CARTESIAN_POINT ( 'NONE',  ( -73.47956238811100604, -286.6642240893996245, -202.6595034932258272 ) ) ;
#72613=CARTESIAN_POINT ( 'NONE',  ( -89.09781327979187893, -278.1377930622334702, -321.9440039371183389 ) ) ;
#72614=CARTESIAN_POINT ( 'NONE',  ( 23.77428276502948634, -293.0922129019433555, -316.6896097107490959 ) ) ;
#72615=CARTESIAN_POINT ( 'NONE',  ( -81.49623364921241375, -284.2866546808349995, -333.3837363610172133 ) ) ;
#72616=CARTESIAN_POINT ( 'NONE',  ( 38.94664176403490075, -283.0307116320295791, -267.0678165391638572 ) ) ;
#72617=CARTESIAN_POINT ( 'NONE',  ( -5.460401608448171906, -282.9773602660387155, -340.4277084256985972 ) ) ;
#72618=CARTESIAN_POINT ( 'NONE',  ( 34.58718658791602962, -281.7194969011699186, -257.7784814298119613 ) ) ;
#72619=CARTESIAN_POINT ( 'NONE',  ( 161.5212002755277751, 220.3141551401068625, -205.3533786008646302 ) ) ;
#72620=CARTESIAN_POINT ( 'NONE',  ( 178.9682605196512952, 254.2604872615934539, -166.3201451735521914 ) ) ;
#72621=CARTESIAN_POINT ( 'NONE',  ( 83.45820220953470425, 82.29232363724392485, -299.0340934522332645 ) ) ;
#72622=CARTESIAN_POINT ( 'NONE',  ( -71.97516272200695653, -272.7793929792926519, -205.8599289353179529 ) ) ;
#72623=CARTESIAN_POINT ( 'NONE',  ( -79.44853104573034841, -295.1121907953627215, -334.7547643554154888 ) ) ;
#72624=CARTESIAN_POINT ( 'NONE',  ( -11.83151317020731952, -92.77902702723882555, -356.4673753601988437 ) ) ;
#72626=CARTESIAN_POINT ( 'NONE',  ( -4.025619730384383921, -273.1671643557605762, -201.4748118082759163 ) ) ;
#72627=CARTESIAN_POINT ( 'NONE',  ( -110.5776835635761017, -298.2551015922192619, -282.5001546655709603 ) ) ;
#72629=CARTESIAN_POINT ( 'NONE',  ( -0.7313374559675888120, -289.8705152877921023, -334.1450890153101341 ) ) ;
#72631=CARTESIAN_POINT ( 'NONE',  ( -50.41561929555482635, -296.1562796411411682, -346.0580913715991755 ) ) ;
#72632=CARTESIAN_POINT ( 'NONE',  ( -81.52076531793906611, -285.9245920000120122, -212.1700650584869550 ) ) ;
#72633=CARTESIAN_POINT ( 'NONE',  ( -92.93856628502165051, -272.1975345855373121, -217.5169543012414408 ) ) ;
#72634=CARTESIAN_POINT ( 'NONE',  ( 39.49414499237111187, -294.3182804409632354, -267.4325367030131702 ) ) ;
#72635=CARTESIAN_POINT ( 'NONE',  ( 37.72526998099149864, -294.2563479062197302, -287.2870475415577971 ) ) ;
#72636=CARTESIAN_POINT ( 'NONE',  ( -87.93212010360555553, -291.4876291612071100, -217.6641788733667227 ) ) ;
#72638=CARTESIAN_POINT ( 'NONE',  ( -43.94181038247550930, -275.8896270874741958, -195.0376113436787762 ) ) ;
#72639=CARTESIAN_POINT ( 'NONE',  ( 35.35801304190726313, -274.0397283439281182, -246.0533773938741149 ) ) ;
#72641=CARTESIAN_POINT ( 'NONE',  ( -112.3403395174902357, -278.2746858806543742, -253.1933868178968794 ) ) ;
#72642=CARTESIAN_POINT ( 'NONE',  ( 36.44315350027425637, -273.9325050280429537, -268.8658627906413017 ) ) ;
#72643=CARTESIAN_POINT ( 'NONE',  ( -43.52183335250149554, -275.0520673500969338, -197.2620434942434144 ) ) ;
#72644=CARTESIAN_POINT ( 'NONE',  ( 26.97912606564017679, -276.9711285845758084, -305.4848690527435338 ) ) ;
#72645=CARTESIAN_POINT ( 'NONE',  ( -40.42847179124874657, -299.6142133325463988, -194.1720776783739950 ) ) ;
#72646=CARTESIAN_POINT ( 'NONE',  ( 17.68453685504397299, -274.2898273730569940, -321.8443195779528310 ) ) ;
#72647=CARTESIAN_POINT ( 'NONE',  ( -102.8558341196655732, -296.7631799731530577, -302.9068089170913254 ) ) ;
#72648=CARTESIAN_POINT ( 'NONE',  ( -41.08721893353986587, -293.6749017781283442, -343.8676367511934018 ) ) ;
#72650=CARTESIAN_POINT ( 'NONE',  ( -111.2798458314029659, -279.3114653483224856, -249.0848985517635583 ) ) ;
#72651=CARTESIAN_POINT ( 'NONE',  ( 19.85417795680242392, -275.0783346835104339, -224.9799936443723425 ) ) ;
#72652=CARTESIAN_POINT ( 'NONE',  ( -82.96826716633719911, -284.1275919621877506, -208.8824062727275077 ) ) ;
#72653=CARTESIAN_POINT ( 'NONE',  ( -104.8775391835034014, -298.9863765758392447, -237.3620442603397578 ) ) ;
#72655=CARTESIAN_POINT ( 'NONE',  ( -99.74171250033620595, -284.2756170267631433, -232.0698491973785735 ) ) ;
#72656=CARTESIAN_POINT ( 'NONE',  ( -109.7608660887781014, -276.5932177258724209, -285.6398096063447838 ) ) ;
#72657=CARTESIAN_POINT ( 'NONE',  ( -21.54408018272725300, -275.4204838017519137, -342.2870973895800262 ) ) ;
#72659=CARTESIAN_POINT ( 'NONE',  ( -4.491375455754583967, -284.6194807504754181, -337.7980639928842379 ) ) ;
#72660=CARTESIAN_POINT ( 'NONE',  ( 35.01452081217395573, -276.5946514338101565, -257.9695860609151623 ) ) ;
#72661=ADVANCED_FACE ( 'NONE', ( #69387 ), #39819, .T. ) ;
#72663=CARTESIAN_POINT ( 'NONE',  ( 37.94046176882081056, -273.8019471926983783, -258.4854946276341821 ) ) ;
#72665=CARTESIAN_POINT ( 'NONE',  ( -74.13335367105617024, -281.5645111751994136, -204.8141679600256850 ) ) ;
#72667=CARTESIAN_POINT ( 'NONE',  ( 18.57537894557212610, -290.1762498905588359, -321.1996306617678556 ) ) ;
#72668=CARTESIAN_POINT ( 'NONE',  ( 24.30966394850093693, -292.1314378457955740, -313.0929279872260054 ) ) ;
#72670=CARTESIAN_POINT ( 'NONE',  ( -65.71210231118379852, -296.4675217324693790, -202.6687935621388306 ) ) ;
#72671=CARTESIAN_POINT ( 'NONE',  ( -73.20321590351130681, -289.7113434673329380, -205.3047678917250494 ) ) ;
#72672=CARTESIAN_POINT ( 'NONE',  ( -111.8439089875458023, -277.9397250554267202, -284.5643135594219189 ) ) ;
#72673=CARTESIAN_POINT ( 'NONE',  ( -67.60359018049207691, -295.6549983607338845, -201.7233188019406782 ) ) ;
#72674=CARTESIAN_POINT ( 'NONE',  ( -15.17234992714933561, -287.2501807962000839, -343.4316190599973879 ) ) ;
#72675=CARTESIAN_POINT ( 'NONE',  ( -2.028130870471564151, -284.1764967702965805, -335.1782835905693787 ) ) ;
#72676=CARTESIAN_POINT ( 'NONE',  ( -49.16465440331155889, -284.1434735829894294, -195.2468375549695452 ) ) ;
#72677=CARTESIAN_POINT ( 'NONE',  ( -6.994032904470032896, -284.0712237367500848, -337.4151858539075874 ) ) ;
#72678=CARTESIAN_POINT ( 'NONE',  ( -80.71366044929442296, -284.4601327357931950, -329.3433649550614746 ) ) ;
#72679=CARTESIAN_POINT ( 'NONE',  ( -106.2175352299979494, -292.1319217335318967, -301.0593786139695567 ) ) ;
#72680=CARTESIAN_POINT ( 'NONE',  ( -38.36138943496778353, -274.3729763839149314, -193.3890157287981708 ) ) ;
#72681=CARTESIAN_POINT ( 'NONE',  ( -110.5333982167679778, -288.3920446292280531, -289.1823228490201814 ) ) ;
#72682=CARTESIAN_POINT ( 'NONE',  ( -102.0969893335362002, -278.0044214041092800, -312.1207748972948934 ) ) ;
#72683=CARTESIAN_POINT ( 'NONE',  ( 19.23523255358808726, -296.2103464493407046, -319.0724779203311527 ) ) ;
#72684=LINE ( 'NONE', #87333, #86292 ) ;
#72686=CARTESIAN_POINT ( 'NONE',  ( -48.41943294058848579, -281.8809335630779174, -343.0145921786399299 ) ) ;
#72687=CARTESIAN_POINT ( 'NONE',  ( -111.2673279605176759, -276.3768176437554303, -284.0345360605514315 ) ) ;
#72688=CARTESIAN_POINT ( 'NONE',  ( -112.3828400292837273, -271.2102467711956137, -256.2397729456131401 ) ) ;
#72689=CARTESIAN_POINT ( 'NONE',  ( -5.028484675708946305, -275.9637644424725522, -335.9474968275684432 ) ) ;
#72690=CARTESIAN_POINT ( 'NONE',  ( -64.34350742637757037, -293.2134153304747883, -201.7791664698164595 ) ) ;
#72691=CARTESIAN_POINT ( 'NONE',  ( 32.97945695563360857, -294.7636269776970153, -290.8596603395666307 ) ) ;
#72692=CARTESIAN_POINT ( 'NONE',  ( 38.26613518709703499, -294.8337160385650009, -258.9585248358236527 ) ) ;
#72693=CARTESIAN_POINT ( 'NONE',  ( 31.79163058365386973, -295.2913694723740150, -303.2547929590451190 ) ) ;
#72694=CARTESIAN_POINT ( 'NONE',  ( -100.1675541633565132, -295.8734854955789046, -307.6347335298187318 ) ) ;
#72695=CARTESIAN_POINT ( 'NONE',  ( -15.23856689835864664, -290.7662682545058601, -342.0844431101372720 ) ) ;
#72696=CARTESIAN_POINT ( 'NONE',  ( -99.78723085027833406, -284.1204814658040050, -315.5008100114276317 ) ) ;
#72697=CARTESIAN_POINT ( 'NONE',  ( -64.43587502152126945, -271.8418671105007434, -199.5925777300951722 ) ) ;
#72698=CARTESIAN_POINT ( 'NONE',  ( -35.14611011754089986, -285.9122939627697519, -193.3792836050163260 ) ) ;
#72699=CARTESIAN_POINT ( 'NONE',  ( -46.07608554803450573, -279.1432289929468311, -344.5449098422316752 ) ) ;
#72700=CARTESIAN_POINT ( 'NONE',  ( -99.93999509964166350, -283.8734386798907394, -231.9422072200140406 ) ) ;
#72701=CARTESIAN_POINT ( 'NONE',  ( -109.6215082978459634, -288.2945442657234594, -290.3768613297563661 ) ) ;
#72702=CARTESIAN_POINT ( 'NONE',  ( -22.77999168687133391, -278.3760220647245092, -195.9554462355543194 ) ) ;
#72703=CARTESIAN_POINT ( 'NONE',  ( -78.59295187722810283, -208.2960365483323244, -357.4574221067172743 ) ) ;
#72704=CARTESIAN_POINT ( 'NONE',  ( -105.6202170683752541, -284.4066648466970832, -244.3604917212543910 ) ) ;
#72705=CARTESIAN_POINT ( 'NONE',  ( 12.72102239935743562, -281.9376762649483226, -212.3806684269877110 ) ) ;
#72706=CARTESIAN_POINT ( 'NONE',  ( -75.55697911132457989, -288.6078432237277980, -336.9374851502971069 ) ) ;
#72707=CARTESIAN_POINT ( 'NONE',  ( -51.14747050546461793, -278.8259245745310864, -345.3000338929620057 ) ) ;
#72708=CARTESIAN_POINT ( 'NONE',  ( -39.92938971463601661, -278.3991618759394555, -346.8371776259054968 ) ) ;
#72709=CARTESIAN_POINT ( 'NONE',  ( -57.11117175625147269, -279.6232099540412719, -200.0890182841114893 ) ) ;
#72710=CARTESIAN_POINT ( 'NONE',  ( -94.18229758850212363, -275.2052107901574800, -221.9575668034076728 ) ) ;
#72711=CARTESIAN_POINT ( 'NONE',  ( 22.20925851149811692, -292.8966693147658589, -221.5483806580962209 ) ) ;
#72712=CARTESIAN_POINT ( 'NONE',  ( -81.39817350995882350, -287.6742818801649264, -330.6821868511964340 ) ) ;
#72713=CARTESIAN_POINT ( 'NONE',  ( -99.39157657486194353, -292.7442151106627648, -226.1315662186328552 ) ) ;
#72714=CARTESIAN_POINT ( 'NONE',  ( -108.6027320246684269, -295.2457476494138291, -287.6214016828461126 ) ) ;
#72715=CARTESIAN_POINT ( 'NONE',  ( 34.73549899882192449, -293.0634980774637484, -258.5797030023960588 ) ) ;
#72716=CARTESIAN_POINT ( 'NONE',  ( -81.76257180806857150, -292.5423133271952452, -207.8448907438060758 ) ) ;
#72717=CARTESIAN_POINT ( 'NONE',  ( 33.85778561786663943, -281.9852975541580804, -253.7922949074904579 ) ) ;
#72718=CARTESIAN_POINT ( 'NONE',  ( -36.53081718739017703, -296.9824153312136445, -193.6703720887663280 ) ) ;
#72719=CARTESIAN_POINT ( 'NONE',  ( -26.15118692841940984, -289.5646579613576819, -346.4405843363378494 ) ) ;
#72720=CARTESIAN_POINT ( 'NONE',  ( -78.50876869752676157, -281.7396319832358813, -333.9659758506107892 ) ) ;
#72721=EDGE_CURVE ( 'NONE', #16234, #41846, #64101, .T. ) ;
#72722=CARTESIAN_POINT ( 'NONE',  ( -74.41341025751604832, -289.8645498355145378, -337.8404730962463987 ) ) ;
#72723=CARTESIAN_POINT ( 'NONE',  ( -74.73458058308284535, -285.8727505285902453, -207.6406270880269460 ) ) ;
#72725=CARTESIAN_POINT ( 'NONE',  ( 191.9735245738955882, 278.3896920391067056, -124.9451965857499545 ) ) ;
#72726=CARTESIAN_POINT ( 'NONE',  ( 201.7739257888548252, 292.3635967676956398, -68.22063874808750938 ) ) ;
#72728=CARTESIAN_POINT ( 'NONE',  ( -89.58173318462191048, -278.4898060840101834, -219.0684315871032197 ) ) ;
#72729=CARTESIAN_POINT ( 'NONE',  ( -59.81537445235002082, -278.6745003950895807, -200.5282240395157771 ) ) ;
#72730=CARTESIAN_POINT ( 'NONE',  ( -0.05196895205309185611, -274.2010611771019626, -203.0020846880323404 ) ) ;
#72731=CARTESIAN_POINT ( 'NONE',  ( -81.44234294714043187, -220.1383413502173880, -350.5104082359922586 ) ) ;
#72733=CARTESIAN_POINT ( 'NONE',  ( -67.11599319349446091, -278.2441150999017623, -199.9899749891582417 ) ) ;
#72734=CARTESIAN_POINT ( 'NONE',  ( -93.81978916493524423, -281.8920391718664860, -319.1870551757857015 ) ) ;
#72735=CARTESIAN_POINT ( 'NONE',  ( -3.657551686419955761, -296.3739910336841490, -338.4883214400276188 ) ) ;
#72736=CARTESIAN_POINT ( 'NONE',  ( -98.35438193625856229, -291.6025410122605876, -230.0766589644921680 ) ) ;
#72737=CARTESIAN_POINT ( 'NONE',  ( -45.43326582176418071, -287.8416417169724468, -343.4074734170818601 ) ) ;
#72738=CARTESIAN_POINT ( 'NONE',  ( -5.164482450790024437, -275.1160748727232885, -200.5188711000733122 ) ) ;
#72739=CARTESIAN_POINT ( 'NONE',  ( -93.94119895680513821, -296.0660350180558567, -316.4838732051413217 ) ) ;
#72742=CARTESIAN_POINT ( 'NONE',  ( -112.7927560803320830, -280.4206131454601518, -274.4172677843751558 ) ) ;
#72743=CARTESIAN_POINT ( 'NONE',  ( -1.828323632045869118, -281.6141527805297642, -206.2282390209307721 ) ) ;
#72744=CARTESIAN_POINT ( 'NONE',  ( -112.2958742488556823, -280.1540801664331752, -282.8449393693487650 ) ) ;
#72745=CARTESIAN_POINT ( 'NONE',  ( -18.68723514664256413, -281.8648372545962388, -341.2333140471280331 ) ) ;
#72746=CARTESIAN_POINT ( 'NONE',  ( 12.02521229381300572, -273.2329020383918987, -215.5784457234925640 ) ) ;
#72749=CARTESIAN_POINT ( 'NONE',  ( 18.79224306375114040, -277.0721031080080365, -322.8314833540257496 ) ) ;
#72751=CARTESIAN_POINT ( 'NONE',  ( 33.82390975394172727, -277.2444477822796216, -246.5236143311895489 ) ) ;
#72752=CARTESIAN_POINT ( 'NONE',  ( -51.22351806067383251, -275.8010109056640999, -345.5003315948738418 ) ) ;
#72755=CARTESIAN_POINT ( 'NONE',  ( -109.1111539952250951, -286.2364724873730779, -293.3721318079574871 ) ) ;
#72756=CARTESIAN_POINT ( 'NONE',  ( -7.194386846226396237, -291.6552219792573624, -203.6997256379168277 ) ) ;
#72757=CARTESIAN_POINT ( 'NONE',  ( 33.76833694114049678, -286.5267394708469055, -240.9529536600720974 ) ) ;
#72758=CARTESIAN_POINT ( 'NONE',  ( -109.7156170244136888, -282.5896632547243712, -285.9130119237511849 ) ) ;
#72759=CARTESIAN_POINT ( 'NONE',  ( -80.99010622357680234, -282.2323864183447881, -329.6713975624234081 ) ) ;
#72760=CARTESIAN_POINT ( 'NONE',  ( 32.33085845630967725, -285.2872847148469191, -244.0038636518765145 ) ) ;
#72761=CARTESIAN_POINT ( 'NONE',  ( -8.323208108905429725, -283.8685871247024011, -337.7781605352935230 ) ) ;
#72762=CARTESIAN_POINT ( 'NONE',  ( -13.66897461514133383, -272.3592773133695459, -199.1950957955571937 ) ) ;
#72763=CARTESIAN_POINT ( 'NONE',  ( -93.31806661614903931, -283.6640859793865843, -218.5819076144867665 ) ) ;
#72764=CARTESIAN_POINT ( 'NONE',  ( -112.1286995360680265, -298.6331651887081193, -264.0644008026904999 ) ) ;
#72765=CARTESIAN_POINT ( 'NONE',  ( -64.91578699423818932, -280.6241501027257073, -202.5151292883427629 ) ) ;
#72766=CARTESIAN_POINT ( 'NONE',  ( -88.65379263049631220, -287.3348173322237358, -215.3621891257582774 ) ) ;
#72769=CARTESIAN_POINT ( 'NONE',  ( 35.68445224958905726, -295.2241710157894090, -250.9077759206547285 ) ) ;
#72770=CARTESIAN_POINT ( 'NONE',  ( -77.44622426448674446, -275.5895855807585804, -333.7990799351396163 ) ) ;
#72771=CARTESIAN_POINT ( 'NONE',  ( -57.25892217699154685, -288.4998490426477247, -344.6283936932735514 ) ) ;
#72772=CARTESIAN_POINT ( 'NONE',  ( 33.51259369878102490, -292.2226569974388326, -291.0489143048235974 ) ) ;
#72773=CARTESIAN_POINT ( 'NONE',  ( -109.5308292116296087, -277.0555008853965546, -284.2107635596270256 ) ) ;
#72774=CARTESIAN_POINT ( 'NONE',  ( -111.2782920302880001, -294.7851883511885376, -263.1566089504992760 ) ) ;
#72775=CARTESIAN_POINT ( 'NONE',  ( -41.63830181620294013, -293.3122229488282073, -196.9434854874232599 ) ) ;
#72776=CARTESIAN_POINT ( 'NONE',  ( -4.829096099716510437, -276.9805209788416391, -202.7746430608542312 ) ) ;
#72777=CARTESIAN_POINT ( 'NONE',  ( -76.74098044987496792, -294.0489582041214476, -335.7709305526648222 ) ) ;
#72778=CARTESIAN_POINT ( 'NONE',  ( 34.79696273316833555, -289.3561883829402177, -285.9913912323960972 ) ) ;
#72779=CARTESIAN_POINT ( 'NONE',  ( -110.5714814780118047, -288.5345247329788094, -290.6434536131768596 ) ) ;
#72780=CARTESIAN_POINT ( 'NONE',  ( 14.51133573259076925, -289.7301019903147790, -322.5783334252406007 ) ) ;
#72782=CARTESIAN_POINT ( 'NONE',  ( -98.23942683986632574, -290.7930844619075401, -310.9310364460142182 ) ) ;
#72784=CARTESIAN_POINT ( 'NONE',  ( -7.062681113594275750, -289.8687120359217033, -340.7399770864576567 ) ) ;
#72785=CARTESIAN_POINT ( 'NONE',  ( -14.69747092412048595, -278.3641297292050467, -198.4339793144716850 ) ) ;
#72786=CARTESIAN_POINT ( 'NONE',  ( -82.22996982939004340, -279.7913096560416193, -207.8248282407932663 ) ) ;
#72788=CARTESIAN_POINT ( 'NONE',  ( 25.91053145502498722, -281.7988824034962363, -314.2579755673482964 ) ) ;
#72789=CARTESIAN_POINT ( 'NONE',  ( 37.68168330610299677, -285.5252883469739231, -268.2817470021191752 ) ) ;
#72790=DIRECTION ( 'NONE',  ( 0.000000000000000000, 0.000000000000000000, 1.000000000000000000 ) ) ;
#72791=CARTESIAN_POINT ( 'NONE',  ( 14.20963097909127804, -278.9248101955988659, -216.8729293222980061 ) ) ;
#72792=CARTESIAN_POINT ( 'NONE',  ( -89.07745193319594534, -281.7789361043462009, -324.7316401023517756 ) ) ;
#72794=CARTESIAN_POINT ( 'NONE',  ( -105.7326466465223263, -276.5917805852744209, -304.3236144910305825 ) ) ;
#72795=CARTESIAN_POINT ( 'NONE',  ( -93.68326502999310890, -284.1844589753897026, -218.2533082595517442 ) ) ;
#72796=CARTESIAN_POINT ( 'NONE',  ( -40.54020606039571106, -298.9522361910534869, -197.1831134738568494 ) ) ;
#72797=CARTESIAN_POINT ( 'NONE',  ( -80.00965940080263294, -293.0645425674039757, -210.0831407724429027 ) ) ;
#72798=CARTESIAN_POINT ( 'NONE',  ( -3.697203440359453364, -299.7802514347591227, -193.8469198602112442 ) ) ;
#72799=CARTESIAN_POINT ( 'NONE',  ( 32.53538869069117823, -275.4999698196624536, -291.6006793084644073 ) ) ;
#72800=CARTESIAN_POINT ( 'NONE',  ( -12.31756191903461328, -296.7269406582806823, -341.1179870220809107 ) ) ;
#72801=CARTESIAN_POINT ( 'NONE',  ( -97.28873851984336341, -290.0707921930952011, -318.7073966601080883 ) ) ;
#72802=CARTESIAN_POINT ( 'NONE',  ( 37.00423617923385677, -279.8048493502550400, -283.9234460782151359 ) ) ;
#72803=CARTESIAN_POINT ( 'NONE',  ( 26.49409145742661664, -292.8170659981735753, -227.2093164448088487 ) ) ;
#72804=CARTESIAN_POINT ( 'NONE',  ( -96.75650345722364420, -289.0140461432455368, -313.1780491418830366 ) ) ;
#72805=CARTESIAN_POINT ( 'NONE',  ( -5.378620047332675291, -292.6314885091609312, -338.2232907747255126 ) ) ;
#72808=CARTESIAN_POINT ( 'NONE',  ( -110.4291984882819406, -290.0849398905399994, -268.4539024029337497 ) ) ;
#72810=CARTESIAN_POINT ( 'NONE',  ( -73.51277607011510895, -286.5258270450058262, -202.5935002401162421 ) ) ;
#72811=CARTESIAN_POINT ( 'NONE',  ( -67.74223827176244583, -294.1233781216987495, -207.3071070584150277 ) ) ;
#72812=CARTESIAN_POINT ( 'NONE',  ( -4.613761650278911830, -293.6902255782867428, -339.8140205573930075 ) ) ;
#72813=CARTESIAN_POINT ( 'NONE',  ( 4.291474855843541825, -283.8189811163575769, -334.6107874504319284 ) ) ;
#72814=CARTESIAN_POINT ( 'NONE',  ( -95.76466535220404808, -284.9998614853337244, -226.5917549651722140 ) ) ;
#72815=CARTESIAN_POINT ( 'NONE',  ( 22.67393365139516703, -276.2789273492726352, -227.9203913018577055 ) ) ;
#72816=CARTESIAN_POINT ( 'NONE',  ( -39.76718585308042719, -293.1028433265271929, -344.9792155617773233 ) ) ;
#72817=CARTESIAN_POINT ( 'NONE',  ( 36.09587323923904023, -274.3634149236244184, -271.6069373902695361 ) ) ;
#72819=EDGE_CURVE ( 'NONE', #64529, #85520, #61379, .T. ) ;
#72821=CARTESIAN_POINT ( 'NONE',  ( -0.7199747513541546740, -294.2460677926919743, -338.0856253332792676 ) ) ;
#72822=CARTESIAN_POINT ( 'NONE',  ( 33.19748600952929962, -289.1624936713531611, -246.5800873834269282 ) ) ;
#72823=CARTESIAN_POINT ( 'NONE',  ( -109.5644004111295402, -297.9587339726267601, -244.5662721191335436 ) ) ;
#72824=CARTESIAN_POINT ( 'NONE',  ( 30.05252867172026043, -287.8225472969218117, -241.9120375200736817 ) ) ;
#72825=EDGE_CURVE ( 'NONE', #48357, #64930, #56517, .T. ) ;
#72826=CARTESIAN_POINT ( 'NONE',  ( -112.4847428916724112, -277.8085886051226225, -254.6024475216803751 ) ) ;
#72827=CARTESIAN_POINT ( 'NONE',  ( -81.80599152132158736, -296.2913906368955850, -333.1656076759642815 ) ) ;
#72828=CARTESIAN_POINT ( 'NONE',  ( -70.12637761404209868, -287.6189855326091447, -338.6796219301734254 ) ) ;
#72829=CARTESIAN_POINT ( 'NONE',  ( -107.1454133446231793, -296.4699679027177694, -302.8139439399148500 ) ) ;
#72830=CARTESIAN_POINT ( 'NONE',  ( -4.827476657401152060, -292.8258111386011251, -204.9643726217158246 ) ) ;
#72833=CARTESIAN_POINT ( 'NONE',  ( 161.3931422173053249, 217.5860020223464630, -202.5160790843344500 ) ) ;
#72834=CARTESIAN_POINT ( 'NONE',  ( 11.61776537017173183, -288.2371227443646831, -211.7628872388046659 ) ) ;
#72835=CARTESIAN_POINT ( 'NONE',  ( -37.30987171927208834, -289.5523547857346784, -190.3611179825600175 ) ) ;
#72837=CARTESIAN_POINT ( 'NONE',  ( -17.01094650526230012, -279.6565829699431447, -196.1993135046544978 ) ) ;
#72838=CARTESIAN_POINT ( 'NONE',  ( -81.69270557300031044, -285.6572679393446492, -330.7000851468633300 ) ) ;
#72839=CARTESIAN_POINT ( 'NONE',  ( -104.9025625061584464, -283.5926130349020582, -234.5528345699403303 ) ) ;
#72840=CARTESIAN_POINT ( 'NONE',  ( 22.31309839122275207, -286.2449531403032097, -314.9090593353636223 ) ) ;
#72841=CARTESIAN_POINT ( 'NONE',  ( 19.09960526085329136, -276.7151387656413135, -219.7401610571842241 ) ) ;
#72842=CARTESIAN_POINT ( 'NONE',  ( -81.98667224417084753, -297.9173867170221683, -212.4626196692436793 ) ) ;
#72843=CARTESIAN_POINT ( 'NONE',  ( 21.71281251067375351, -292.8462644033361926, -314.1082094983529487 ) ) ;
#72844=CARTESIAN_POINT ( 'NONE',  ( -96.74399494036289582, -279.8605757033813006, -221.5074523464344054 ) ) ;
#72845=CARTESIAN_POINT ( 'NONE',  ( -51.28088489548370177, -277.2353657018302897, -342.0179329272686459 ) ) ;
#72846=CARTESIAN_POINT ( 'NONE',  ( -109.7215378930284544, -278.0403781914830006, -259.7606838162875533 ) ) ;
#72847=CARTESIAN_POINT ( 'NONE',  ( -32.71504482354093568, -275.1888127968763342, -193.7968178094361349 ) ) ;
#72848=CARTESIAN_POINT ( 'NONE',  ( -48.46280659700573779, -276.1107419331834194, -346.2950548609296106 ) ) ;
#72849=CARTESIAN_POINT ( 'NONE',  ( -95.90218042510922203, -239.8047343563239906, -341.6332487328612615 ) ) ;
#72850=CARTESIAN_POINT ( 'NONE',  ( -35.06784298841319725, -275.0234667435146321, -345.3392106192002302 ) ) ;
#72852=CARTESIAN_POINT ( 'NONE',  ( -113.1920869093001585, -298.0938358568027979, -261.1239583833628330 ) ) ;
#72853=CARTESIAN_POINT ( 'NONE',  ( 21.31550574532285580, -278.6948066931273615, -317.0979686699210447 ) ) ;
#72855=CARTESIAN_POINT ( 'NONE',  ( 65.71450562203199297, 45.78484130816451625, -315.1169351998001389 ) ) ;
#72857=CARTESIAN_POINT ( 'NONE',  ( -79.49822820460157402, -286.5477384608152533, -210.3233512628877691 ) ) ;
#72858=CARTESIAN_POINT ( 'NONE',  ( -100.1714248532217084, -286.8844126864483997, -227.5317330673458116 ) ) ;
#72859=CARTESIAN_POINT ( 'NONE',  ( 2.509519063279600282, -285.9506782573768646, -209.0767562171938039 ) ) ;
#72860=CARTESIAN_POINT ( 'NONE',  ( -110.7015735226289479, -276.8410931493526164, -278.8619500997134537 ) ) ;
#72861=CARTESIAN_POINT ( 'NONE',  ( -100.0621680825726116, -285.8717648333191050, -310.1688694095292362 ) ) ;
#72862=CARTESIAN_POINT ( 'NONE',  ( -92.71675402643796815, -277.7197443720456249, -221.7177449714219790 ) ) ;
#72863=CARTESIAN_POINT ( 'NONE',  ( -37.79611087004261094, -278.3731007715740020, -343.8654030349177901 ) ) ;
#72864=CARTESIAN_POINT ( 'NONE',  ( 33.64781523500835192, -276.2728844942318460, -287.6903298064727323 ) ) ;
#72865=CARTESIAN_POINT ( 'NONE',  ( 39.24340640033333472, -286.3263062569518524, -268.7087937074405204 ) ) ;
#72867=CARTESIAN_POINT ( 'NONE',  ( 3.727008315224979551, -281.3922982625654186, -205.3558374599040235 ) ) ;
#72868=CARTESIAN_POINT ( 'NONE',  ( 31.02533418221001682, -282.4997674295435104, -305.6524132644659062 ) ) ;
#72871=ADVANCED_FACE ( 'NONE', ( #11156, #40017 ), #3120, .T. ) ;
#72872=DIRECTION ( 'NONE',  ( -5.501794166262391869E-14, -0.01273136352371387336, 0.9999189529070978688 ) ) ;
#72873=CARTESIAN_POINT ( 'NONE',  ( -36.08321065769175817, -290.8969748645503728, -346.1283686582925725 ) ) ;
#72874=CARTESIAN_POINT ( 'NONE',  ( -104.1710195045417606, -289.7229458616542956, -233.1167849466729649 ) ) ;
#72875=CARTESIAN_POINT ( 'NONE',  ( -33.45504803521652804, -296.6041469108583328, -346.4749179285185505 ) ) ;
#72876=CARTESIAN_POINT ( 'NONE',  ( -41.86814187491255268, -297.1908200787846113, -197.3397988196830397 ) ) ;
#72877=CARTESIAN_POINT ( 'NONE',  ( -11.18011930742364690, -291.7327735019198371, -197.9941258714229377 ) ) ;
#72878=CARTESIAN_POINT ( 'NONE',  ( 22.56642320430477611, -285.4368467842198811, -227.3597378230043091 ) ) ;
#72879=CARTESIAN_POINT ( 'NONE',  ( 21.50096932750649970, -289.3696776354869939, -314.2532319823305897 ) ) ;
#72880=CARTESIAN_POINT ( 'NONE',  ( -69.91165696735023971, -288.1233781216987495, -202.8022627189028810 ) ) ;
#72881=CARTESIAN_POINT ( 'NONE',  ( -2.701219136153005351, -290.5942469076187535, -336.8820750439425069 ) ) ;
#72882=CARTESIAN_POINT ( 'NONE',  ( -81.78955137494219230, -287.6558560713782526, -330.9780870856083652 ) ) ;
#72883=CARTESIAN_POINT ( 'NONE',  ( -68.83941802020008538, -291.4663706477062988, -338.4403842650248180 ) ) ;
#72884=CARTESIAN_POINT ( 'NONE',  ( -103.7037371727642494, -285.9117644680385979, -239.2652485834057927 ) ) ;
#72885=CARTESIAN_POINT ( 'NONE',  ( -109.8706853286312963, -292.8061080240303227, -250.5745675780537454 ) ) ;
#72888=CARTESIAN_POINT ( 'NONE',  ( -106.5764924421242199, -274.9207630375488520, -240.4809386914803326 ) ) ;
#72889=CARTESIAN_POINT ( 'NONE',  ( -38.89874539361407102, -282.2693099806596138, -343.5185427964374298 ) ) ;
#72890=CARTESIAN_POINT ( 'NONE',  ( -23.72675424202179428, -280.8779958886743771, -344.1149917413332560 ) ) ;
#72891=CARTESIAN_POINT ( 'NONE',  ( 30.75450656246835734, -293.2095365323900751, -305.9569808653699283 ) ) ;
#72892=CARTESIAN_POINT ( 'NONE',  ( -47.36141293730224788, -296.3227172363077671, -197.1926891426785460 ) ) ;
#72893=CARTESIAN_POINT ( 'NONE',  ( 21.96974492092504860, -274.2519511699902637, -315.3440779453779328 ) ) ;
#72894=CARTESIAN_POINT ( 'NONE',  ( -102.9802714674142408, -298.3143374500106688, -237.1899057006374392 ) ) ;
#72896=CARTESIAN_POINT ( 'NONE',  ( -85.76700008427775401, -293.9519832235627064, -328.9184773446665986 ) ) ;
#72897=CARTESIAN_POINT ( 'NONE',  ( -8.987206350759501916, -296.0991782222057509, -338.2821074093562288 ) ) ;
#72898=DIRECTION ( 'NONE',  ( -1.000000000000000000, -0.000000000000000000, -0.000000000000000000 ) ) ;
#72899=CARTESIAN_POINT ( 'NONE',  ( -80.24121609794639198, -296.4529576600072005, -329.6252155125271770 ) ) ;
#72900=DIRECTION ( 'NONE',  ( -0.8510748438184358999, -0.5250018354872690862, -0.006684530980050039546 ) ) ;
#72902=CARTESIAN_POINT ( 'NONE',  ( -36.55668731188109177, -284.0820710801025371, -194.9972418441998911 ) ) ;
#72903=CARTESIAN_POINT ( 'NONE',  ( -108.2990148797109384, -296.3252440394299470, -287.5619941437095690 ) ) ;
#72904=CARTESIAN_POINT ( 'NONE',  ( -80.93820472494256535, -285.4784231988035685, -206.8275166316477680 ) ) ;
#72905=CARTESIAN_POINT ( 'NONE',  ( -8.564236707468705134, -284.5987463175507628, -340.2819924957438502 ) ) ;
#72906=CARTESIAN_POINT ( 'NONE',  ( 27.42470994676389395, -287.7659505920086076, -312.0653609268888431 ) ) ;
#72907=CARTESIAN_POINT ( 'NONE',  ( 21.64331529827405021, -290.9185876760646465, -224.2882593392528179 ) ) ;
#72908=CARTESIAN_POINT ( 'NONE',  ( -35.32998854785326159, -279.2739403521234749, -193.5358233559415453 ) ) ;
#72909=CARTESIAN_POINT ( 'NONE',  ( -95.99890600148557951, -275.4094976428775681, -317.0979686699210447 ) ) ;
#72911=CARTESIAN_POINT ( 'NONE',  ( 33.05514607539908667, -286.0731952119183461, -249.5462283535254358 ) ) ;
#72912=CARTESIAN_POINT ( 'NONE',  ( -80.37856714471620023, -288.5403802820315491, -333.9022088773372161 ) ) ;
#72913=CARTESIAN_POINT ( 'NONE',  ( 129.9467878515196162, -299.5541904835127980, -195.3611179825600175 ) ) ;
#72914=CARTESIAN_POINT ( 'NONE',  ( -101.5916249803873228, -279.4294639178291391, -311.8164708445809765 ) ) ;
#72915=CARTESIAN_POINT ( 'NONE',  ( 32.90881567044437617, -291.9252086300456313, -297.6241301183516157 ) ) ;
#72916=CARTESIAN_POINT ( 'NONE',  ( 34.08676926968254861, -281.0180828953170362, -255.1337540159136950 ) ) ;
#72917=CARTESIAN_POINT ( 'NONE',  ( 4.229085249920590428, -294.6753844772217121, -335.2380124001516037 ) ) ;
#72918=CARTESIAN_POINT ( 'NONE',  ( 17.32686730478499015, -284.9045123526669272, -218.1256683838033155 ) ) ;
#72920=CARTESIAN_POINT ( 'NONE',  ( -110.5270659326031790, -280.3417573866738053, -286.7593765964139720 ) ) ;
#72921=CARTESIAN_POINT ( 'NONE',  ( -108.2002714205350316, -295.3667624903945352, -288.9167126970091317 ) ) ;
#72926=CARTESIAN_POINT ( 'NONE',  ( 35.04456948638337366, -283.2962415486646250, -252.0863400165810333 ) ) ;
#72928=CARTESIAN_POINT ( 'NONE',  ( -106.6662871844225293, -293.6237833571632336, -303.7098442033569086 ) ) ;
#72929=CARTESIAN_POINT ( 'NONE',  ( 26.01722170459059669, -274.1741510155194419, -226.8658954243709616 ) ) ;
#72931=CARTESIAN_POINT ( 'NONE',  ( -108.4269854908923065, -290.6053003448192271, -253.6969092170724878 ) ) ;
#72933=CARTESIAN_POINT ( 'NONE',  ( -1.647042530098138169, -282.0545322102891532, -205.8894251845867700 ) ) ;
#72934=CARTESIAN_POINT ( 'NONE',  ( -98.51764879670965058, -274.7208677167836868, -228.9910603197111243 ) ) ;
#72935=CARTESIAN_POINT ( 'NONE',  ( 26.06759514603298200, -283.7143089214390557, -312.6186816612479333 ) ) ;
#72936=CARTESIAN_POINT ( 'NONE',  ( 33.33769916781566423, -280.6071985825294632, -290.1488167041902670 ) ) ;
#72937=CARTESIAN_POINT ( 'NONE',  ( -109.1491514686639874, -280.8312899128474101, -248.7118551419337678 ) ) ;
#72938=CARTESIAN_POINT ( 'NONE',  ( 19.38870777905117748, -298.7440530408346717, -193.3610971472934636 ) ) ;
#72940=CARTESIAN_POINT ( 'NONE',  ( -78.83976814825660995, -273.3426100920561339, -205.5004183633851653 ) ) ;
#72941=CARTESIAN_POINT ( 'NONE',  ( 28.75412573992997878, -295.0156052494062351, -236.1170528349503002 ) ) ;
#72945=CARTESIAN_POINT ( 'NONE',  ( 33.29126716111535700, -292.0446656426726690, -297.7707770550896385 ) ) ;
#72946=CARTESIAN_POINT ( 'NONE',  ( -92.06009166544629352, -272.7509353165534094, -221.9474208573190879 ) ) ;
#72947=CARTESIAN_POINT ( 'NONE',  ( -33.59296365779650984, -293.6186511641000152, -194.1465870286367874 ) ) ;
#72948=CARTESIAN_POINT ( 'NONE',  ( -20.25526795762937127, -282.7662352645560304, -195.3538533559490702 ) ) ;
#72949=CARTESIAN_POINT ( 'NONE',  ( -7.359831313354650462, -293.6417368952126594, -199.8550546068382232 ) ) ;
#72950=CARTESIAN_POINT ( 'NONE',  ( -75.63264206588554828, -291.5644342603516748, -334.6710555069792576 ) ) ;
#72951=CARTESIAN_POINT ( 'NONE',  ( 33.83424821312373609, -273.8510802730876890, -293.4698350415559389 ) ) ;
#72952=CARTESIAN_POINT ( 'NONE',  ( -0.7413004339061621817, -278.4825690187726082, -335.2401704488314635 ) ) ;
#72953=CARTESIAN_POINT ( 'NONE',  ( -8.698964420001162878, -292.7542922301141743, -339.0838532300561496 ) ) ;
#72954=CARTESIAN_POINT ( 'NONE',  ( 7.791421277713025617, -282.5211529432661450, -209.4411152510967327 ) ) ;
#72955=CARTESIAN_POINT ( 'NONE',  ( -97.55219031966049670, -283.6428974568090098, -311.7624974560998794 ) ) ;
#72956=CARTESIAN_POINT ( 'NONE',  ( 3.645104413674261412, -281.6690924702567145, -205.4788437199935629 ) ) ;
#72957=CARTESIAN_POINT ( 'NONE',  ( -16.26589251418299753, -281.5806564344613889, -344.0626971093176962 ) ) ;
#72958=CARTESIAN_POINT ( 'NONE',  ( -51.25816404865174292, -278.1671542396359200, -345.8538477270203089 ) ) ;
#72961=CARTESIAN_POINT ( 'NONE',  ( 36.95535874902696349, -276.8520650188337413, -252.9073650446686656 ) ) ;
#72962=CARTESIAN_POINT ( 'NONE',  ( 7.399455738971494334, -289.1948066931273615, -214.2051214447836571 ) ) ;
#72964=CARTESIAN_POINT ( 'NONE',  ( -61.17494723188499250, -299.7430216201950657, -199.1937522017736626 ) ) ;
#72965=CARTESIAN_POINT ( 'NONE',  ( -36.47174376346121250, -275.0613415323690560, -345.0136011372182452 ) ) ;
#72966=CARTESIAN_POINT ( 'NONE',  ( -44.81992495491951445, -293.7190018679248737, -194.6911018076216351 ) ) ;
#72967=CARTESIAN_POINT ( 'NONE',  ( 32.72916948474068022, -292.6233481988778635, -249.3547692446408632 ) ) ;
#72968=CARTESIAN_POINT ( 'NONE',  ( 38.04673431516613391, -287.2521329936142251, -285.7270170991233158 ) ) ;
#72970=CARTESIAN_POINT ( 'NONE',  ( 36.51774155373829700, -291.8792854290135210, -250.7302646962422159 ) ) ;
#72971=CARTESIAN_POINT ( 'NONE',  ( -45.75063976348201322, -281.5602377114073533, -343.7320429426130772 ) ) ;
#72972=CARTESIAN_POINT ( 'NONE',  ( -105.1667797009182976, -292.0115798283595723, -300.6645239998105126 ) ) ;
#72973=CARTESIAN_POINT ( 'NONE',  ( -109.6636208144652898, -282.8471098087292148, -284.5120028395191412 ) ) ;
#72974=CARTESIAN_POINT ( 'NONE',  ( 12.26179021644768596, -283.6593451517005064, -324.5896826196237726 ) ) ;
#72975=CARTESIAN_POINT ( 'NONE',  ( -93.41270723345925830, -290.7755172703175504, -322.8673070979820636 ) ) ;
#72976=CARTESIAN_POINT ( 'NONE',  ( 35.41300954710498416, -281.9493111653811184, -263.1390325155098253 ) ) ;
#72977=CARTESIAN_POINT ( 'NONE',  ( 36.32654883532413947, -292.0819357405638925, -249.3133399081882828 ) ) ;
#72978=CARTESIAN_POINT ( 'NONE',  ( 38.39595957079421851, -288.1915868864134609, -257.3236137424045751 ) ) ;
#72979=CARTESIAN_POINT ( 'NONE',  ( 38.91344462144095928, -287.9164386581488202, -260.1298031878205279 ) ) ;
#72980=CARTESIAN_POINT ( 'NONE',  ( -71.18010625531486824, -285.7589915692370823, -205.6775630764324205 ) ) ;
#72983=CARTESIAN_POINT ( 'NONE',  ( 37.59834304831932883, -295.5542698966260104, -281.5099030915685034 ) ) ;
#72984=CARTESIAN_POINT ( 'NONE',  ( -39.11331488911429943, -293.7587814665974406, -346.8474543798751029 ) ) ;
#72986=CARTESIAN_POINT ( 'NONE',  ( -99.66167402074758286, -278.1407705060379953, -231.7984487048651090 ) ) ;
#72987=CARTESIAN_POINT ( 'NONE',  ( -26.21970324939029595, -297.5365650024917841, -193.4642417802111822 ) ) ;
#72988=CARTESIAN_POINT ( 'NONE',  ( 34.63110557976099102, -291.8243916359490413, -254.4716231057545031 ) ) ;
#72989=CARTESIAN_POINT ( 'NONE',  ( -4.883618958754046169, -276.2456833634645932, -203.8305878720648252 ) ) ;
#72990=CARTESIAN_POINT ( 'NONE',  ( -96.90263219420342011, -295.3996471118767886, -226.4026223922836323 ) ) ;
#72992=CARTESIAN_POINT ( 'NONE',  ( 35.23294904900917146, -294.9053319230876014, -281.6489240585741527 ) ) ;
#72993=CARTESIAN_POINT ( 'NONE',  ( 22.83384010455815982, -294.0504229666166225, -228.4686050845659224 ) ) ;
#72996=CARTESIAN_POINT ( 'NONE',  ( -100.1116814962002763, -293.9939406137900164, -311.8069342023820241 ) ) ;
#72997=CARTESIAN_POINT ( 'NONE',  ( -46.44614785560266768, -275.9367614351162956, -195.9157710565602031 ) ) ;
#72998=CARTESIAN_POINT ( 'NONE',  ( -84.82851503168700447, -290.6668188310470100, -326.1811687410632885 ) ) ;
#72999=CARTESIAN_POINT ( 'NONE',  ( -35.64586920953354365, -295.3636096911404252, -343.3750672587078157 ) ) ;
#73001=CARTESIAN_POINT ( 'NONE',  ( -110.1485337288108894, -280.7812182887895460, -250.8800308435527597 ) ) ;
#73002=CARTESIAN_POINT ( 'NONE',  ( -90.70213895787689751, -277.9998595718899992, -215.4606255731293629 ) ) ;
#73004=CARTESIAN_POINT ( 'NONE',  ( 25.97822374580684013, -275.4786133166169861, -314.0869707326524463 ) ) ;
#73005=CARTESIAN_POINT ( 'NONE',  ( -91.81150306074128764, -281.9165261843410804, -321.0992177375026699 ) ) ;
#73006=CARTESIAN_POINT ( 'NONE',  ( -112.9208981838525574, -277.0797625313704771, -260.2535643847490974 ) ) ;
#73007=CARTESIAN_POINT ( 'NONE',  ( -69.16251303111366155, -277.6344828261087514, -202.2481427452304104 ) ) ;
#73008=CARTESIAN_POINT ( 'NONE',  ( -86.41723836161217775, -296.0382991430520860, -215.6543083155183922 ) ) ;
#73009=CARTESIAN_POINT ( 'NONE',  ( 16.79684297403802518, -278.2820851640076398, -322.3382056213806663 ) ) ;
#73011=CARTESIAN_POINT ( 'NONE',  ( -97.86808708340419116, -289.1823146644446183, -225.4511688677434620 ) ) ;
#73012=CARTESIAN_POINT ( 'NONE',  ( -114.3901258662136797, -290.5413011400655137, -271.2287573755081667 ) ) ;
#73013=CARTESIAN_POINT ( 'NONE',  ( -52.20854811850352206, -275.8625448284764730, -196.6261857251957963 ) ) ;
#73014=CARTESIAN_POINT ( 'NONE',  ( -112.3417001281295313, -270.5523135751785162, -270.3357089863371812 ) ) ;
#73015=CARTESIAN_POINT ( 'NONE',  ( -110.5348553077014344, -283.4541966234602910, -293.7908656783237120 ) ) ;
#73017=CARTESIAN_POINT ( 'NONE',  ( -77.91273765620854874, -283.5073216542049863, -207.2213837150852100 ) ) ;
#73020=CARTESIAN_POINT ( 'NONE',  ( -3.439277640331756647, -291.3051705249692418, -205.2630668959616287 ) ) ;
#73021=CARTESIAN_POINT ( 'NONE',  ( -42.74071489663341339, -284.1229211537595347, -196.3096664007881600 ) ) ;
#73024=CARTESIAN_POINT ( 'NONE',  ( 12.27242766794423723, -290.7420802497326804, -214.0473386744183983 ) ) ;
#73025=CARTESIAN_POINT ( 'NONE',  ( -107.8752399937672379, -279.8657679334177715, -292.2452165140078364 ) ) ;
#73026=CARTESIAN_POINT ( 'NONE',  ( -24.58451979740540594, -284.0980321384393505, -345.9481484084293470 ) ) ;
#73027=CARTESIAN_POINT ( 'NONE',  ( 18.79075021819331326, -274.3319095723495593, -320.9617173160100947 ) ) ;
#73028=CARTESIAN_POINT ( 'NONE',  ( -81.47857639685697961, -285.4323240396813617, -212.2152999623895084 ) ) ;
#73029=CARTESIAN_POINT ( 'NONE',  ( -110.7476787434561203, -280.0453493713906710, -265.1710101379803177 ) ) ;
#73030=CARTESIAN_POINT ( 'NONE',  ( 15.72202112586517941, -277.0794065282693737, -320.7282026081434196 ) ) ;
#73032=CARTESIAN_POINT ( 'NONE',  ( -109.0223123248972144, -286.8388378420689833, -248.1205266937496958 ) ) ;
#73034=CARTESIAN_POINT ( 'NONE',  ( -111.9109958098805038, -270.5893608454304058, -270.3361269473657558 ) ) ;
#73035=CARTESIAN_POINT ( 'NONE',  ( -100.0097404549985640, -295.7918157752228581, -315.1914770268384700 ) ) ;
#73036=CARTESIAN_POINT ( 'NONE',  ( 36.14531818545879815, -289.7009962858164727, -283.4571075966876492 ) ) ;
#73038=CARTESIAN_POINT ( 'NONE',  ( 13.79469577742117714, -277.1948066931273047, -206.1857440867352693 ) ) ;
#73039=CARTESIAN_POINT ( 'NONE',  ( -88.71415407399018704, -278.2710857511310678, -213.4193627885387343 ) ) ;
#73040=CARTESIAN_POINT ( 'NONE',  ( 36.67798197893209533, -292.1814147632391041, -288.5133634305834107 ) ) ;
#73041=CARTESIAN_POINT ( 'NONE',  ( -5.516593998334935023, -287.9986249842356756, -203.8801421112974026 ) ) ;
#73042=CARTESIAN_POINT ( 'NONE',  ( -79.65225891650069912, -281.2316758307698024, -209.6339360414947635 ) ) ;
#73043=CARTESIAN_POINT ( 'NONE',  ( 36.93595832552122005, -289.2040309470683610, -288.3450775158492547 ) ) ;
#73044=CARTESIAN_POINT ( 'NONE',  ( -59.51578583863269500, -285.3393142978532637, -342.0628349263005248 ) ) ;
#73045=CARTESIAN_POINT ( 'NONE',  ( -80.22442354794887365, -277.7818054746463758, -334.3789732546630376 ) ) ;
#73046=CARTESIAN_POINT ( 'NONE',  ( -104.8482221143613913, -270.9780595289846019, -238.0671880161435467 ) ) ;
#73047=CARTESIAN_POINT ( 'NONE',  ( 36.36221646880999714, -291.4192034941190173, -253.6582961215340788 ) ) ;
#73048=CARTESIAN_POINT ( 'NONE',  ( -101.8900607146500192, -278.9379215109555616, -228.2823930435663158 ) ) ;
#73050=CARTESIAN_POINT ( 'NONE',  ( -90.13700449647819823, -275.1563556530194319, -218.1737505820852903 ) ) ;
#73052=CARTESIAN_POINT ( 'NONE',  ( -4.829096099716510437, -288.9805209788416391, -202.7746430608542312 ) ) ;
#73053=CARTESIAN_POINT ( 'NONE',  ( 6.666607923622994925, -272.8809367692422825, -208.3510484586181235 ) ) ;
#73056=CARTESIAN_POINT ( 'NONE',  ( -85.52006280609499811, -278.8718443071332445, -215.4354062334244588 ) ) ;
#73058=CARTESIAN_POINT ( 'NONE',  ( 38.98616187440877923, -276.8387606310905653, -276.8469641047298637 ) ) ;
#73059=CARTESIAN_POINT ( 'NONE',  ( -86.50733033714197973, -298.7783042571975898, -215.6060659608170909 ) ) ;
#73060=CARTESIAN_POINT ( 'NONE',  ( -81.43623256062613791, -282.6942458828311828, -333.2628231212455603 ) ) ;
#73061=CARTESIAN_POINT ( 'NONE',  ( 34.06544669660750202, -289.5681981683001140, -290.0192744247504493 ) ) ;
#73062=CARTESIAN_POINT ( 'NONE',  ( -26.35364258250954705, -299.7074747675757749, -194.0516646480180896 ) ) ;
#73063=CARTESIAN_POINT ( 'NONE',  ( -101.9895631524544939, -298.2986125637458485, -229.2677788079590186 ) ) ;
#73064=CARTESIAN_POINT ( 'NONE',  ( -12.37311779704040759, -296.7269406588296761, -340.9607307062144628 ) ) ;
#73065=CARTESIAN_POINT ( 'NONE',  ( 36.02311296814248465, -279.7426621485017790, -285.1778750019664699 ) ) ;
#73067=CARTESIAN_POINT ( 'NONE',  ( -95.03391018387637246, -271.2286763439871606, -222.9760077353333827 ) ) ;
#73068=CARTESIAN_POINT ( 'NONE',  ( 17.75877964030828338, -288.4242270669927279, -217.6506670674926909 ) ) ;
#73069=CARTESIAN_POINT ( 'NONE',  ( -53.48993985878833257, -288.1845432221370515, -341.8695820006565214 ) ) ;
#73070=CARTESIAN_POINT ( 'NONE',  ( -98.66049953969873343, -248.8406155931078274, -334.2579121867940444 ) ) ;
#73072=CARTESIAN_POINT ( 'NONE',  ( -8.472701289815535830, -287.2563324886975238, -341.1226210832681431 ) ) ;
#73073=CARTESIAN_POINT ( 'NONE',  ( 32.33251146571912216, -287.5104289021707586, -292.3832470775842012 ) ) ;
#73075=CARTESIAN_POINT ( 'NONE',  ( -80.77451170167559269, -286.5579207549085936, -207.0903385480012560 ) ) ;
#73077=CARTESIAN_POINT ( 'NONE',  ( 11.76506004665075089, -276.6811842291739367, -324.4724358216403175 ) ) ;
#73078=CARTESIAN_POINT ( 'NONE',  ( 1.555230137263102996, -291.4792703585474669, -204.2056330633209598 ) ) ;
#73079=CARTESIAN_POINT ( 'NONE',  ( 35.51518249018909756, -282.5156972125018910, -295.1272094515709341 ) ) ;
#73080=CARTESIAN_POINT ( 'NONE',  ( 26.15577599719389923, -283.6343154095646355, -312.6787062672458433 ) ) ;
#73081=CARTESIAN_POINT ( 'NONE',  ( -24.53291955609521580, -283.2263779232612819, -346.3209468134538156 ) ) ;
#73082=CARTESIAN_POINT ( 'NONE',  ( 33.78001832583415620, -281.6672170382085483, -253.8145578856452289 ) ) ;
#73083=CARTESIAN_POINT ( 'NONE',  ( -99.62977921489535049, -248.4066214194129714, -334.3629173841853799 ) ) ;
#73084=CARTESIAN_POINT ( 'NONE',  ( -68.78513416746625353, -279.4665886414322813, -338.2820478901094816 ) ) ;
#73085=CARTESIAN_POINT ( 'NONE',  ( 120.6115914165433622, 149.8424774028926549, -263.0264761077845037 ) ) ;
#73086=CARTESIAN_POINT ( 'NONE',  ( 4.580739421786890198, -58.54268714549175456, -351.3897242287694667 ) ) ;
#73088=CARTESIAN_POINT ( 'NONE',  ( -107.3480541873074117, -272.0321835944646978, -248.9341396886358382 ) ) ;
#73089=CARTESIAN_POINT ( 'NONE',  ( 37.03546872130033307, -293.3064656943403747, -290.0477544997108907 ) ) ;
#73090=CARTESIAN_POINT ( 'NONE',  ( -101.5192183512151018, -254.7299117250532277, -324.2986292072765764 ) ) ;
#73091=CARTESIAN_POINT ( 'NONE',  ( -107.6178393504614377, -271.6262271496485710, -239.9854724940879294 ) ) ;
#73092=CARTESIAN_POINT ( 'NONE',  ( -98.78793098692258923, -288.3905111404708919, -311.2595676259820721 ) ) ;
#73093=CARTESIAN_POINT ( 'NONE',  ( -58.74205432471467958, -297.1923203538758003, -341.4448033007763570 ) ) ;
#73094=CARTESIAN_POINT ( 'NONE',  ( 21.57882386082837556, -289.4797581162507072, -314.3095773604123337 ) ) ;
#73095=EDGE_LOOP ( 'NONE', ( #81564, #54280, #9743, #93411 ) ) ;
#73096=CARTESIAN_POINT ( 'NONE',  ( -76.95051930630967263, -296.5099352471046927, -336.1797910864050891 ) ) ;
#73097=CARTESIAN_POINT ( 'NONE',  ( 9.064752347471532801, -287.2018323135091578, -213.9303674108047915 ) ) ;
#73098=CARTESIAN_POINT ( 'NONE',  ( -10.44309843443351049, -273.3152305445330512, -198.4856947690159359 ) ) ;
#73100=CARTESIAN_POINT ( 'NONE',  ( -2.032560889525590664, -295.3994176685293951, -338.6064365563865408 ) ) ;
#73102=CARTESIAN_POINT ( 'NONE',  ( 36.22629968212283558, -293.7614618421599175, -247.8383227035716914 ) ) ;
#73103=CARTESIAN_POINT ( 'NONE',  ( -107.0022520373381241, -291.0086096485084113, -248.4922429912959672 ) ) ;
#73105=CARTESIAN_POINT ( 'NONE',  ( -57.75651281168471485, -275.7108350334418674, -197.5568130899085304 ) ) ;
#73106=CARTESIAN_POINT ( 'NONE',  ( 38.92354293375725405, -274.2499612741542023, -262.6357259258361410 ) ) ;
#73109=CARTESIAN_POINT ( 'NONE',  ( -114.3161071221565095, -278.0802304824414932, -268.7292890590784964 ) ) ;
#73110=CARTESIAN_POINT ( 'NONE',  ( 14.06839398099382699, -273.1885869972965111, -217.4135718842441918 ) ) ;
#73111=CARTESIAN_POINT ( 'NONE',  ( -92.25880484591469610, -274.3226999491774905, -221.7983989117779231 ) ) ;
#73112=CARTESIAN_POINT ( 'NONE',  ( -85.47380000771069319, -274.3088133280386387, -215.0965126812099868 ) ) ;
#73113=CARTESIAN_POINT ( 'NONE',  ( -93.41286672215939291, -275.0192372706783317, -219.0583908918939358 ) ) ;
#73114=CARTESIAN_POINT ( 'NONE',  ( 9.483832685155217490, -274.4325049931520653, -329.4681939319050343 ) ) ;
#73115=CARTESIAN_POINT ( 'NONE',  ( -93.15485587731009787, -296.5333459091953614, -317.5905093728383690 ) ) ;
#73116=CARTESIAN_POINT ( 'NONE',  ( 21.78919188548751507, -292.7361839201291218, -314.1665118064395301 ) ) ;
#73118=CARTESIAN_POINT ( 'NONE',  ( -34.28725712780541102, -277.5070560793624850, -347.2389254522084343 ) ) ;
#73119=CARTESIAN_POINT ( 'NONE',  ( 35.69887234250364827, -275.7349499831626076, -271.5828482630395797 ) ) ;
#73120=CARTESIAN_POINT ( 'NONE',  ( -93.54599913363162500, -283.9489943653851469, -218.3761255032945598 ) ) ;
#73121=CARTESIAN_POINT ( 'NONE',  ( -95.96129336208792893, -297.9062562753256884, -317.4322159043396141 ) ) ;
#73124=CARTESIAN_POINT ( 'NONE',  ( -39.96950239376612046, -285.2154572861724660, -197.2468486323607522 ) ) ;
#73125=CARTESIAN_POINT ( 'NONE',  ( -101.4719067437793001, -276.2911120056779737, -307.4139430091987037 ) ) ;
#73126=CARTESIAN_POINT ( 'NONE',  ( -103.6699102018617538, -276.6977129306728784, -302.3529546323155728 ) ) ;
#73127=CARTESIAN_POINT ( 'NONE',  ( -72.40716872195855558, -285.5163125606239873, -336.6733609061362813 ) ) ;
#73128=CARTESIAN_POINT ( 'NONE',  ( 28.39292233211522998, -277.1989220997525649, -303.1267739309547551 ) ) ;
#73130=CARTESIAN_POINT ( 'NONE',  ( 7.751075117740841236, -274.8481405682493914, -331.8518526148474166 ) ) ;
#73132=CARTESIAN_POINT ( 'NONE',  ( -96.27574277624613330, -281.1918237722447316, -223.7048531446321249 ) ) ;
#73134=CARTESIAN_POINT ( 'NONE',  ( -0.4412112234383363529, -288.4587809395545719, -204.4095045454016031 ) ) ;
#73137=CARTESIAN_POINT ( 'NONE',  ( 6.758878966034807867, -290.6513980749826374, -209.6336831662218856 ) ) ;
#73139=CARTESIAN_POINT ( 'NONE',  ( 9.260745600255551935, -297.4432165736817524, -196.9738530863085089 ) ) ;
#73140=CARTESIAN_POINT ( 'NONE',  ( -44.39435959057286141, -290.1017168606732071, -196.4100128921299984 ) ) ;
#73141=CARTESIAN_POINT ( 'NONE',  ( -101.7183354143585632, -264.3591293023451385, -316.7762957234928649 ) ) ;
#73143=CARTESIAN_POINT ( 'NONE',  ( -57.12993618525803896, -287.7826750952785346, -344.1119553580791148 ) ) ;
#73144=CARTESIAN_POINT ( 'NONE',  ( 20.82394529270771599, -283.7855490092647415, -315.7835585854966780 ) ) ;
#73145=CARTESIAN_POINT ( 'NONE',  ( -43.56068242780591504, -284.2146047317261264, -194.5768080435144327 ) ) ;
#73148=CARTESIAN_POINT ( 'NONE',  ( -0.9449166246075736408, -283.9840292369245844, -334.3193001659674337 ) ) ;
#73149=CARTESIAN_POINT ( 'NONE',  ( -107.5127507160505900, -285.6304174285627937, -249.4820569209224743 ) ) ;
#73150=CARTESIAN_POINT ( 'NONE',  ( -95.11347048095392154, -291.8664548480630287, -318.7632418221128887 ) ) ;
#73151=CARTESIAN_POINT ( 'NONE',  ( -68.83929638076644153, -273.9825625775587241, -200.1068109098702053 ) ) ;
#73153=CARTESIAN_POINT ( 'NONE',  ( 15.65814368809771295, -286.3895567345195445, -324.2885693897821398 ) ) ;
#73154=CARTESIAN_POINT ( 'NONE',  ( 23.51804566061516510, -276.1822351590183189, -317.5533758655669203 ) ) ;
#73155=CARTESIAN_POINT ( 'NONE',  ( 36.53202046756055665, -295.3939881498735076, -259.6597064731944897 ) ) ;
#73157=CARTESIAN_POINT ( 'NONE',  ( -37.30987171927208124, -291.5519495502701943, -345.3611179825600175 ) ) ;
#73158=CARTESIAN_POINT ( 'NONE',  ( -65.52016485367887810, -282.1132798393017538, -338.2512978017085175 ) ) ;
#73160=CARTESIAN_POINT ( 'NONE',  ( -110.9176308258383159, -276.7498517870059231, -254.9169901867596195 ) ) ;
#73163=CARTESIAN_POINT ( 'NONE',  ( -106.2090945444642358, -271.4571733933473752, -237.4979206764600406 ) ) ;
#73164=CARTESIAN_POINT ( 'NONE',  ( 34.72754688294035930, -274.7384623431737509, -258.0426876069348054 ) ) ;
#73165=CARTESIAN_POINT ( 'NONE',  ( -2.124973169838737963, -294.0473952654028267, -205.6127962383809518 ) ) ;
#73167=CARTESIAN_POINT ( 'NONE',  ( 27.68999468555567844, -294.0368607340075755, -236.6819387010903881 ) ) ;
#73168=CARTESIAN_POINT ( 'NONE',  ( -108.3579801980407211, -286.0397047751482660, -291.2548693938053361 ) ) ;
#73169=CARTESIAN_POINT ( 'NONE',  ( -25.13360142715051992, -293.6301744186044971, -194.9318887829286950 ) ) ;
#73170=CARTESIAN_POINT ( 'NONE',  ( 34.98090694058139860, -294.5489106884811008, -245.2461233633605673 ) ) ;
#73171=CARTESIAN_POINT ( 'NONE',  ( -82.36147831468070990, -295.5194750967788195, -327.8905101744839499 ) ) ;
#73172=CARTESIAN_POINT ( 'NONE',  ( -31.69606010021917797, -290.9811823337887517, -345.2003426393226846 ) ) ;
#73173=CARTESIAN_POINT ( 'NONE',  ( -79.15794535491855299, -283.7664013229027091, -335.0171435302522696 ) ) ;
#73174=CARTESIAN_POINT ( 'NONE',  ( 29.23053802437308946, -296.9591603901928352, -194.8226834078566299 ) ) ;
#73175=CARTESIAN_POINT ( 'NONE',  ( -52.17120467166177633, -285.7007987483117404, -194.7482356052953776 ) ) ;
#73176=CARTESIAN_POINT ( 'NONE',  ( -111.8072690319441733, -280.4562987191866910, -276.2328196184652143 ) ) ;
#73177=CARTESIAN_POINT ( 'NONE',  ( -77.25217553056639019, -284.2992028870982608, -208.7030595633969199 ) ) ;
#73178=CARTESIAN_POINT ( 'NONE',  ( 36.58979311425390080, -285.3890465491662098, -257.6705470108576037 ) ) ;
#73179=CARTESIAN_POINT ( 'NONE',  ( -108.4387400044720522, -277.0297852208477707, -244.0274134981911516 ) ) ;
#73180=CARTESIAN_POINT ( 'NONE',  ( 196.7445862410842778, 294.2657832282549748, -82.73034305482168804 ) ) ;
#73181=CARTESIAN_POINT ( 'NONE',  ( -109.5601635404877499, -283.9096509625210842, -281.7530366059522180 ) ) ;
#73182=CARTESIAN_POINT ( 'NONE',  ( 37.86193009706390455, -282.5740009459709086, -255.7863891489984951 ) ) ;
#73183=CARTESIAN_POINT ( 'NONE',  ( -97.11444395950869080, -288.9630396228041036, -318.5486378931654485 ) ) ;
#73184=CARTESIAN_POINT ( 'NONE',  ( 14.35554667347608415, -277.9402894807163875, -326.4136181273895545 ) ) ;
#73185=CARTESIAN_POINT ( 'NONE',  ( -31.47128582580520373, -278.2947990966504790, -346.6947026069813091 ) ) ;
#73186=CARTESIAN_POINT ( 'NONE',  ( -37.00619625555646053, -279.8897888413432042, -197.3618889339537361 ) ) ;
#73187=CARTESIAN_POINT ( 'NONE',  ( -84.24320124703196200, -275.3832176796396993, -212.2913668866021055 ) ) ;
#73188=CARTESIAN_POINT ( 'NONE',  ( 38.60628375436721171, -293.7117920417641699, -283.1257928102254482 ) ) ;
#73189=CARTESIAN_POINT ( 'NONE',  ( -53.79507220571837678, -287.2844673148395032, -343.1700003172549600 ) ) ;
#73190=CARTESIAN_POINT ( 'NONE',  ( -83.79495375490245124, -293.0269081422002273, -209.8914931144436764 ) ) ;
#73191=CARTESIAN_POINT ( 'NONE',  ( 34.36707742795692155, -292.6733840335568857, -285.6553619667395196 ) ) ;
#73192=CARTESIAN_POINT ( 'NONE',  ( 32.36572248969818588, -293.5069782880681259, -292.1088240402822862 ) ) ;
#73193=CARTESIAN_POINT ( 'NONE',  ( -113.7004471572712703, -291.7282508814546986, -262.6816388558936524 ) ) ;
#73194=CARTESIAN_POINT ( 'NONE',  ( 29.06180668779334653, -281.7902840199041066, -239.6707851293002136 ) ) ;
#73195=CARTESIAN_POINT ( 'NONE',  ( -43.25215934052818767, -296.8996391772359402, -193.8453268357231991 ) ) ;
#73196=CARTESIAN_POINT ( 'NONE',  ( -71.85327816632135978, -290.1477650267762556, -339.0798473680692950 ) ) ;
#73197=CARTESIAN_POINT ( 'NONE',  ( -92.54800716189920706, -281.9718319951990111, -322.2701159640413948 ) ) ;
#73198=CARTESIAN_POINT ( 'NONE',  ( 32.84733707369120737, -288.2893156450637093, -301.9719286036957442 ) ) ;
#73199=CARTESIAN_POINT ( 'NONE',  ( -72.38788856700459462, -285.9080880295402380, -206.2855813242020986 ) ) ;
#73202=CARTESIAN_POINT ( 'NONE',  ( 197.6688820137005678, 288.5744782996524123, -96.90442113908628130 ) ) ;
#73203=CARTESIAN_POINT ( 'NONE',  ( -21.90833566152406675, -108.8621393979285443, -358.8400048060100858 ) ) ;
#73204=CARTESIAN_POINT ( 'NONE',  ( -107.7709874604358902, -278.0111077307921050, -250.5077099796372408 ) ) ;
#73205=CARTESIAN_POINT ( 'NONE',  ( -109.5930718114085352, -277.3085056103241754, -282.8436747111708769 ) ) ;
#73206=CARTESIAN_POINT ( 'NONE',  ( 13.95354979347750835, -274.4151795074977827, -212.8917841408612048 ) ) ;
#73207=CARTESIAN_POINT ( 'NONE',  ( 66.34501194978001593, 45.89495233920238348, -316.1728383282853656 ) ) ;
#73208=CARTESIAN_POINT ( 'NONE',  ( -113.7879192522227925, -277.1474555070945485, -268.7285821512305688 ) ) ;
#73210=CARTESIAN_POINT ( 'NONE',  ( -1.664197571552678223, -280.5970545489188339, -335.9422017180141893 ) ) ;
#73211=CARTESIAN_POINT ( 'NONE',  ( -19.50312986280587069, -296.5860549155258923, -344.2783976665886030 ) ) ;
#73214=CARTESIAN_POINT ( 'NONE',  ( -49.70530253418396427, -292.3826893828946822, -198.3019032850177155 ) ) ;
#73215=CARTESIAN_POINT ( 'NONE',  ( -63.48825068814020511, -274.6608112161942472, -198.1864818107218298 ) ) ;
#73216=CARTESIAN_POINT ( 'NONE',  ( -80.71194023548018492, -288.3388930672060724, -329.7562829896559151 ) ) ;
#73217=CARTESIAN_POINT ( 'NONE',  ( -114.2397671894842119, -273.2034605398562803, -270.3693937356876518 ) ) ;
#73218=CARTESIAN_POINT ( 'NONE',  ( -108.8842984839512837, -296.5265477094952757, -284.9373756802219191 ) ) ;
#73223=CARTESIAN_POINT ( 'NONE',  ( -79.13504755576629179, -281.4137194915968507, -207.3489146086906203 ) ) ;
#73225=AXIS2_PLACEMENT_3D ( 'NONE', #17566, #10435, #3822 ) ;
#73226=CARTESIAN_POINT ( 'NONE',  ( -3.016480513786325535, -281.5965610198867921, -205.5703009478988008 ) ) ;
#73227=CARTESIAN_POINT ( 'NONE',  ( -103.9166967655488349, -280.7930338330506288, -233.7312963297764270 ) ) ;
#73228=CARTESIAN_POINT ( 'NONE',  ( -62.24596879253420667, -272.2021386847839608, -201.0034568747851438 ) ) ;
#73231=CARTESIAN_POINT ( 'NONE',  ( -59.73565045294212439, -279.9206511083185092, -200.8275204372000928 ) ) ;
#73232=CARTESIAN_POINT ( 'NONE',  ( 12.60741885962485576, -277.1789520242494973, -328.7498526183424588 ) ) ;
#73234=CARTESIAN_POINT ( 'NONE',  ( -3.601420209294212249, -278.6070885727895075, -337.3574602997516081 ) ) ;
#73235=CARTESIAN_POINT ( 'NONE',  ( -67.49293634223286631, -276.0147363679222394, -340.5715819368065240 ) ) ;
#73238=CARTESIAN_POINT ( 'NONE',  ( 37.88885930567494142, -283.5980066611590473, -275.5225696371106210 ) ) ;
#73239=CARTESIAN_POINT ( 'NONE',  ( -28.07578558877671426, -291.3697968209031046, -197.7379168887302967 ) ) ;
#73240=CARTESIAN_POINT ( 'NONE',  ( -4.809520512284307436, -285.8180479359820652, -200.6835026635681629 ) ) ;
#73241=CARTESIAN_POINT ( 'NONE',  ( -111.1075222570720058, -282.7133142886193014, -276.4090513059687169 ) ) ;
#73242=CARTESIAN_POINT ( 'NONE',  ( -18.60297489575357233, -281.3808948384404971, -341.5773804018525652 ) ) ;
#73243=CARTESIAN_POINT ( 'NONE',  ( -10.20263917335970305, -284.4889851876559419, -201.0307626556661091 ) ) ;
#73244=CARTESIAN_POINT ( 'NONE',  ( -64.97978957592825111, -280.8879312464148938, -202.3665114541418006 ) ) ;
#73246=CARTESIAN_POINT ( 'NONE',  ( -96.94180419081259004, -283.5944028192403152, -222.8819855696234242 ) ) ;
#73247=CARTESIAN_POINT ( 'NONE',  ( -27.97177029087859168, -296.9334926536926105, -344.8254258010556441 ) ) ;
#73248=CARTESIAN_POINT ( 'NONE',  ( -97.83645399810694698, -278.9209622056022795, -311.6381479445759055 ) ) ;
#73249=CARTESIAN_POINT ( 'NONE',  ( -112.5204223572541053, -286.5208734570495039, -272.8154048871286932 ) ) ;
#73251=CARTESIAN_POINT ( 'NONE',  ( 115.2448031289451222, -299.5541904835127980, -198.2496582146980302 ) ) ;
#73252=CARTESIAN_POINT ( 'NONE',  ( -69.04176417201057347, -293.5587077001491139, -201.7582674619375780 ) ) ;
#73253=CARTESIAN_POINT ( 'NONE',  ( 1.896654034993785931, -274.5274096662241163, -334.3388897330638656 ) ) ;
#73254=CARTESIAN_POINT ( 'NONE',  ( 27.30339984700533407, -287.2964748890674400, -311.9943683261041087 ) ) ;
#73255=CARTESIAN_POINT ( 'NONE',  ( -6.922078925331913268, -290.8580551372217542, -203.1220886693526211 ) ) ;
#73256=CARTESIAN_POINT ( 'NONE',  ( -105.7327961481518059, -276.8795873496372906, -297.2665349502402705 ) ) ;
#73257=CARTESIAN_POINT ( 'NONE',  ( -78.65652458365705968, -293.7542639725073172, -332.0993964455642526 ) ) ;
#73258=CARTESIAN_POINT ( 'NONE',  ( -74.95399505978609511, -290.8795582832368609, -333.5151035318205004 ) ) ;
#73261=CARTESIAN_POINT ( 'NONE',  ( -95.06977275496491586, -294.3518305742202870, -320.2627951568942990 ) ) ;
#73262=CARTESIAN_POINT ( 'NONE',  ( 16.54482709176679478, -288.4344903114027829, -219.9174554845207012 ) ) ;
#73263=CARTESIAN_POINT ( 'NONE',  ( -95.62838437909911704, -288.1270263401531793, -319.1320661971221284 ) ) ;
#73264=CARTESIAN_POINT ( 'NONE',  ( 16.45401370096022831, -289.6944855736180102, -320.6492043221166455 ) ) ;
#73266=CARTESIAN_POINT ( 'NONE',  ( -110.2827589834297015, -291.2721597052092193, -276.6539497295956380 ) ) ;
#73268=CARTESIAN_POINT ( 'NONE',  ( -57.17322733088074926, -290.5074341996305520, -344.4072813486337736 ) ) ;
#73269=CARTESIAN_POINT ( 'NONE',  ( -53.38516879397450055, -277.8676110552775071, -196.6801831234620010 ) ) ;
#73270=CARTESIAN_POINT ( 'NONE',  ( -14.23815008033865759, -280.6769305874645397, -196.8751976733161939 ) ) ;
#73271=CARTESIAN_POINT ( 'NONE',  ( -14.23006120043628719, -280.0104755763516664, -196.8777411304390625 ) ) ;
#73272=CARTESIAN_POINT ( 'NONE',  ( 35.00453609008011568, -285.8085040041834759, -290.3278874668597496 ) ) ;
#73274=CARTESIAN_POINT ( 'NONE',  ( -66.53397474552238577, -277.8053176888203097, -202.0927518105919489 ) ) ;
#73276=CARTESIAN_POINT ( 'NONE',  ( -109.5723787496062016, -282.2922277454530899, -290.5534362380706739 ) ) ;
#73277=CARTESIAN_POINT ( 'NONE',  ( -110.6395504398199847, -271.5021483123970825, -270.3477634379551660 ) ) ;
#73278=CARTESIAN_POINT ( 'NONE',  ( -113.0805574562855895, -276.9094828927819663, -280.0718888115501954 ) ) ;
#73279=CARTESIAN_POINT ( 'NONE',  ( -91.67426346666579207, -284.2199701833703784, -216.2365850013540864 ) ) ;
#73280=CARTESIAN_POINT ( 'NONE',  ( -90.32057426773499742, -274.0811625408844066, -219.8864625244989384 ) ) ;
#73281=CARTESIAN_POINT ( 'NONE',  ( -63.37354268129882939, -275.1447534770784387, -198.5213694749504327 ) ) ;
#73282=CARTESIAN_POINT ( 'NONE',  ( 32.11698423171890227, -275.5176906991226247, -292.8906242749386593 ) ) ;
#73283=CARTESIAN_POINT ( 'NONE',  ( -76.68613590182987139, -297.5784857714271538, -334.2731698376891245 ) ) ;
#73284=CARTESIAN_POINT ( 'NONE',  ( 3.181940437418188772, -288.6907664074376498, -335.8975896573491582 ) ) ;
#73285=CARTESIAN_POINT ( 'NONE',  ( 22.25183336013190427, -280.2646852086944591, -316.8354894476419190 ) ) ;
#73287=CARTESIAN_POINT ( 'NONE',  ( -40.63029578579246959, -291.8452168153966113, -193.4181941621540091 ) ) ;
#73288=CARTESIAN_POINT ( 'NONE',  ( -107.9558864063967576, -289.3529395009105087, -289.9657638697507309 ) ) ;
#73289=CARTESIAN_POINT ( 'NONE',  ( 27.75276186004279211, -291.0551154088623207, -233.1091158226316509 ) ) ;
#73292=CARTESIAN_POINT ( 'NONE',  ( -109.8513564468808141, -289.9416630509429069, -279.3242749132838867 ) ) ;
#73294=CARTESIAN_POINT ( 'NONE',  ( 21.90092091071948133, -287.8354745835331983, -221.5437843153170832 ) ) ;
#73295=CARTESIAN_POINT ( 'NONE',  ( -6.998514795304313196, -288.9805209788416391, -207.2794874003663779 ) ) ;
#73296=CARTESIAN_POINT ( 'NONE',  ( 25.51507949784165064, -293.1956637955955216, -314.4504294448437349 ) ) ;
#73297=CARTESIAN_POINT ( 'NONE',  ( -38.70684677102161686, -284.3841067151028597, -346.8557887065531986 ) ) ;
#73298=CARTESIAN_POINT ( 'NONE',  ( -105.5641786249488661, -284.7322795454889501, -244.3862564384492941 ) ) ;
#73299=CARTESIAN_POINT ( 'NONE',  ( 34.31083767777736426, -276.6524942850991238, -253.9599627617523083 ) ) ;
#73300=CARTESIAN_POINT ( 'NONE',  ( 36.83860575284516869, -291.6853601666521740, -279.1282048728275527 ) ) ;
#73302=CARTESIAN_POINT ( 'NONE',  ( -67.20508691652135269, -272.4465815549076524, -203.3002892612697678 ) ) ;
#73304=CARTESIAN_POINT ( 'NONE',  ( 168.1488725781630649, 234.1813984995739588, -193.4213935641190858 ) ) ;
#73305=CARTESIAN_POINT ( 'NONE',  ( 35.46503039139748381, -293.5358602183426910, -295.5229250387068305 ) ) ;
#73306=CARTESIAN_POINT ( 'NONE',  ( 26.16677050198359922, -288.9475975164053807, -231.5282922457939776 ) ) ;
#73307=CARTESIAN_POINT ( 'NONE',  ( -112.5880822664892946, -297.8186922332217819, -255.4788516716729987 ) ) ;
#73308=CARTESIAN_POINT ( 'NONE',  ( -49.44656484132194407, -286.5452997819895700, -198.2167944679387404 ) ) ;
#73309=CARTESIAN_POINT ( 'NONE',  ( -112.2574127015945038, -277.4008211540931370, -287.1079452577531583 ) ) ;
#73310=CARTESIAN_POINT ( 'NONE',  ( 0.4975826701656294593, -295.2130402791743222, -337.3202956423671139 ) ) ;
#73311=CARTESIAN_POINT ( 'NONE',  ( -75.06949527116447030, -287.6888276375071882, -336.0643823954877689 ) ) ;
#73312=CARTESIAN_POINT ( 'NONE',  ( 38.30367215542386106, -293.7069653295882858, -256.0950062600824708 ) ) ;
#73313=CARTESIAN_POINT ( 'NONE',  ( -12.25692811675622806, -292.7208376572637576, -201.7299579199793413 ) ) ;
#73314=CARTESIAN_POINT ( 'NONE',  ( 121.3887860922853150, -299.5541904835127980, -195.3611179825600175 ) ) ;
#73315=CARTESIAN_POINT ( 'NONE',  ( 154.0301839823544867, 204.4104515754077056, -214.4894503004110504 ) ) ;
#73316=CARTESIAN_POINT ( 'NONE',  ( -29.55312618109221390, -287.6692180648167323, -194.4529769964728700 ) ) ;
#73317=CARTESIAN_POINT ( 'NONE',  ( 25.22466315766302358, -284.4094976428775112, -220.5068182859052968 ) ) ;
#73320=CARTESIAN_POINT ( 'NONE',  ( -64.69829773598945621, -279.0528829450703370, -198.4375228125011290 ) ) ;
#73321=CARTESIAN_POINT ( 'NONE',  ( 29.80712511043030233, -283.9903010158200800, -303.5100491196825487 ) ) ;
#73322=CARTESIAN_POINT ( 'NONE',  ( -87.58154494375190779, -231.1970665811080607, -346.4935346893788619 ) ) ;
#73323=CARTESIAN_POINT ( 'NONE',  ( -62.98646271852845047, -284.2993606257402348, -198.3822846776303379 ) ) ;
#73324=CARTESIAN_POINT ( 'NONE',  ( 34.46457145140765022, -285.8884975024154187, -290.1780020825075326 ) ) ;
#73325=CARTESIAN_POINT ( 'NONE',  ( 25.88648902800262519, -276.8546588469999392, -228.6178361735904900 ) ) ;
#73326=CARTESIAN_POINT ( 'NONE',  ( -105.8657291402628005, -297.3839266291053605, -244.8686390916215885 ) ) ;
#73327=CARTESIAN_POINT ( 'NONE',  ( -12.85964614132110384, -293.4121405110421392, -339.7102751670778389 ) ) ;
#73328=CARTESIAN_POINT ( 'NONE',  ( -97.62216726411656964, -279.8432949026999381, -222.6161908273719234 ) ) ;
#73329=CARTESIAN_POINT ( 'NONE',  ( -64.33314122881161268, -277.4143151077616380, -338.2415067401982469 ) ) ;
#73330=CARTESIAN_POINT ( 'NONE',  ( -66.12401788427584393, -274.7638433940988421, -199.2620493716995895 ) ) ;
#73331=CARTESIAN_POINT ( 'NONE',  ( -56.85869194969789220, -276.2183105691128731, -344.5818445310513880 ) ) ;
#73332=CARTESIAN_POINT ( 'NONE',  ( 167.6033460893912093, 232.7025357864140460, -192.5994064319566803 ) ) ;
#73333=CARTESIAN_POINT ( 'NONE',  ( 33.81920494783065578, -273.8600055619412501, -294.2092368426298208 ) ) ;
#73334=CARTESIAN_POINT ( 'NONE',  ( -113.7762999216845685, -297.9508232105048933, -272.4717677076108657 ) ) ;
#73335=CARTESIAN_POINT ( 'NONE',  ( 31.98288692825981272, -278.4805209788417528, -303.7098442033569654 ) ) ;
#73337=CARTESIAN_POINT ( 'NONE',  ( -93.50072443926489996, -286.2981365367771218, -223.2401028949195165 ) ) ;
#73338=CARTESIAN_POINT ( 'NONE',  ( -104.8731547512770845, -285.8559955635038250, -305.3108490011269396 ) ) ;
#73339=CARTESIAN_POINT ( 'NONE',  ( -14.52632670182640950, -285.7043010160943481, -200.8576710055064609 ) ) ;
#73340=CARTESIAN_POINT ( 'NONE',  ( -94.23565343474145095, -276.2927183532285085, -317.3864407143046265 ) ) ;
#73341=CARTESIAN_POINT ( 'NONE',  ( -70.74993889211815201, -285.3579607533563376, -336.6682800726266578 ) ) ;
#73342=CARTESIAN_POINT ( 'NONE',  ( -62.52788662254108942, -278.1984073910530810, -201.0514751904430000 ) ) ;
#73343=CARTESIAN_POINT ( 'NONE',  ( -40.50540227777504754, -278.1725066775952655, -343.6144507909678509 ) ) ;
#73345=CARTESIAN_POINT ( 'NONE',  ( -108.5963038186732490, -273.2573449458428172, -254.2127467091688118 ) ) ;
#73346=CARTESIAN_POINT ( 'NONE',  ( -2.472573370753142097, -281.3043528291304938, -201.8752396110628808 ) ) ;
#73347=CARTESIAN_POINT ( 'NONE',  ( 25.88333741668704135, -282.6243774972468259, -314.2262977005315179 ) ) ;
#73351=CARTESIAN_POINT ( 'NONE',  ( 22.86522010551105666, -288.7890748681822402, -224.3460264735121825 ) ) ;
#73352=CARTESIAN_POINT ( 'NONE',  ( -113.8968530000804122, -289.2263387567450650, -271.2064844508544752 ) ) ;
#73353=CARTESIAN_POINT ( 'NONE',  ( -63.12682566572913601, -296.9048343114305908, -201.8405313894990343 ) ) ;
#73354=CARTESIAN_POINT ( 'NONE',  ( -3.358913634876510734, -291.8376574636761234, -201.3648400860364802 ) ) ;
#73355=CARTESIAN_POINT ( 'NONE',  ( 27.63271879142160614, -286.5028567980066327, -305.2408184777386282 ) ) ;
#73356=CARTESIAN_POINT ( 'NONE',  ( 35.09854842600260838, -286.2963819804556920, -283.3143147896302594 ) ) ;
#73357=CARTESIAN_POINT ( 'NONE',  ( -37.29595047966345334, -287.2577785869079889, -196.9515515626052036 ) ) ;
#73358=CARTESIAN_POINT ( 'NONE',  ( 10.59707575819634329, -295.1948066931273615, -210.1954327657594490 ) ) ;
#73359=CARTESIAN_POINT ( 'NONE',  ( -31.94459168598327281, -290.9843433514939761, -345.2178688343421413 ) ) ;
#73360=CARTESIAN_POINT ( 'NONE',  ( -88.26852729870090286, -287.7633390339995572, -325.6466196857214754 ) ) ;
#73361=CARTESIAN_POINT ( 'NONE',  ( -95.15015134527023122, -286.1250771809836237, -225.3786402061973035 ) ) ;
#73362=CARTESIAN_POINT ( 'NONE',  ( -107.0876376419144407, -292.1879274363793115, -298.3884729142890819 ) ) ;
#73365=CARTESIAN_POINT ( 'NONE',  ( -57.70197485341622468, -275.7705635469097274, -197.7543666000710516 ) ) ;
#73367=CARTESIAN_POINT ( 'NONE',  ( -4.265437929646443749, -279.6968935445552233, -205.0895322268834207 ) ) ;
#73368=CARTESIAN_POINT ( 'NONE',  ( -66.10566474741330012, -281.4284039943358380, -339.6400536383988538 ) ) ;
#73369=CARTESIAN_POINT ( 'NONE',  ( -27.77809146484340630, -294.1309511784212987, -346.6553384539989793 ) ) ;
#73370=CARTESIAN_POINT ( 'NONE',  ( -67.44947321883103086, -271.8916058150929871, -202.7343980839995936 ) ) ;
#73371=CARTESIAN_POINT ( 'NONE',  ( -36.47343707306416150, -275.1210699945360716, -344.8087717291236913 ) ) ;
#73372=CARTESIAN_POINT ( 'NONE',  ( -84.40338773409932571, -298.7040647819113133, -213.8460903892598708 ) ) ;
#73373=CARTESIAN_POINT ( 'NONE',  ( 115.2448031289451222, -299.5541904835127980, -195.3611179825600175 ) ) ;
#73374=CARTESIAN_POINT ( 'NONE',  ( -112.5950373509071056, -294.9266693593818900, -259.7358454896262856 ) ) ;
#73375=CARTESIAN_POINT ( 'NONE',  ( 35.79463408042880701, -295.0899757926691223, -278.9615243916762779 ) ) ;
#73378=CLOSED_SHELL ( 'NONE', ( #88963, #12132, #16268, #66192, #39335, #2831, #45593, #39428, #22795, #56383, #12938, #92215, #63881, #7828, #14492, #19720, #72661, #26447, #82116, #3333, #496, #51867, #27761, #44310, #28653, #33680, #54216, #37952, #5274, #65701, #86089, #35486, #38330, #9523, #86734, #34802, #65528, #71229, #72871, #10298, #88140, #7380, #33038, #11031, #93133, #82778, #85965, #4301, #4457, #79803, #75812, #82798, #3005, #38059, #31464, #42947, #91622, #18033, #51751, #50939, #23451, #4778 ) ) ;
#73379=CARTESIAN_POINT ( 'NONE',  ( -31.57946010632110045, -295.7805257696567764, -343.3455473247669261 ) ) ;
#73381=CARTESIAN_POINT ( 'NONE',  ( -82.27446949089110717, -283.4629807521067164, -209.8026517001472087 ) ) ;
#73382=CARTESIAN_POINT ( 'NONE',  ( -109.8044857332493649, -296.4301988708591580, -279.6058443605987804 ) ) ;
#73383=CARTESIAN_POINT ( 'NONE',  ( -113.5993743774286173, -284.4140470798727733, -281.4038888172017323 ) ) ;
#73384=CARTESIAN_POINT ( 'NONE',  ( 37.25030625446895982, -283.6269863695704316, -282.4980855276584180 ) ) ;
#73385=CARTESIAN_POINT ( 'NONE',  ( 28.68259623934678260, -286.7014099627325550, -230.6788079329030552 ) ) ;
#73386=CARTESIAN_POINT ( 'NONE',  ( 18.11349744355580782, -290.8490223214878938, -220.0382006200393903 ) ) ;
#73387=CARTESIAN_POINT ( 'NONE',  ( -113.1999759985792480, -277.7429151515743797, -282.9640846433767933 ) ) ;
#73388=CARTESIAN_POINT ( 'NONE',  ( 35.77081079830085031, -273.2666405000204009, -287.0812184334320705 ) ) ;
#73390=CARTESIAN_POINT ( 'NONE',  ( 19.83412559953331566, -285.6997226897290147, -224.3188636742244171 ) ) ;
#73391=CARTESIAN_POINT ( 'NONE',  ( -65.34700925199277322, -288.3299657512839076, -341.8118834513197157 ) ) ;
#73393=CARTESIAN_POINT ( 'NONE',  ( -95.46946979002640887, -280.6516830769908211, -220.7449602281085390 ) ) ;
#73394=CARTESIAN_POINT ( 'NONE',  ( -16.97616787945061390, -292.8107036458754919, -342.9661946813372992 ) ) ;
#73395=CARTESIAN_POINT ( 'NONE',  ( 33.96014260557003439, -281.4266088303234028, -286.1134101859606176 ) ) ;
#73396=CARTESIAN_POINT ( 'NONE',  ( 22.28798240855449109, -294.3729556434117285, -319.0983544261346196 ) ) ;
#73398=CARTESIAN_POINT ( 'NONE',  ( -58.75610754793071777, -281.7753311534822842, -198.4832785523234122 ) ) ;
#73399=CARTESIAN_POINT ( 'NONE',  ( -90.58651960381676815, -294.8882949058986469, -320.7173387628213277 ) ) ;
#73400=CARTESIAN_POINT ( 'NONE',  ( -111.2605617548323380, -270.7302858429516732, -256.4444337731355859 ) ) ;
#73403=CARTESIAN_POINT ( 'NONE',  ( 37.20990563626141778, -283.5801565885579407, -274.0900424841237850 ) ) ;
#73404=CARTESIAN_POINT ( 'NONE',  ( -107.8934490052756416, -296.3109284114943307, -251.3276888148648993 ) ) ;
#73406=CARTESIAN_POINT ( 'NONE',  ( 21.31550574532286291, -278.4094976428775681, -223.6242672951989618 ) ) ;
#73407=CARTESIAN_POINT ( 'NONE',  ( -3.887150547582444826, -273.6794228174786667, -201.1732918123841500 ) ) ;
#73408=CARTESIAN_POINT ( 'NONE',  ( -107.0009799201558138, -290.6753033575084828, -248.4881913945528140 ) ) ;
#73409=CARTESIAN_POINT ( 'NONE',  ( -108.9680842564292078, -280.2987881553842726, -253.0299653613055568 ) ) ;
#73410=CARTESIAN_POINT ( 'NONE',  ( -66.14395323749488398, -275.2688830278736418, -202.4135600266756398 ) ) ;
#73411=CARTESIAN_POINT ( 'NONE',  ( -4.490082734689728738, -284.2266176671263338, -339.1301797416747377 ) ) ;
#73412=CARTESIAN_POINT ( 'NONE',  ( -2.949519435062557537, -279.3121831882229458, -205.5062231937867523 ) ) ;
#73413=CARTESIAN_POINT ( 'NONE',  ( -77.40317453103840251, -279.5892618867650867, -333.8262779501284854 ) ) ;
#73415=CARTESIAN_POINT ( 'NONE',  ( -58.11957492624920008, -273.6243368184152018, -196.1620496523297561 ) ) ;
#73416=CARTESIAN_POINT ( 'NONE',  ( -92.76125680455017175, -293.1699437487487785, -220.6430816547708105 ) ) ;
#73417=CARTESIAN_POINT ( 'NONE',  ( 121.3395553409046670, -299.5541904835127980, -195.3611179825600175 ) ) ;
#73419=CARTESIAN_POINT ( 'NONE',  ( 37.59135382436164008, -291.8340384855868592, -281.5567825920381324 ) ) ;
#73420=CARTESIAN_POINT ( 'NONE',  ( -40.77155924984348445, -273.5156386562580337, -197.3303878431244129 ) ) ;
#73422=CARTESIAN_POINT ( 'NONE',  ( 6.085613872039532524, -294.1499191793195109, -207.6173840327866174 ) ) ;
#73423=CARTESIAN_POINT ( 'NONE',  ( -85.33152481854864391, -281.9090924074130839, -210.2361428286349110 ) ) ;
#73424=CARTESIAN_POINT ( 'NONE',  ( -19.49426017161818336, -293.4817097101841910, -195.8117653585358653 ) ) ;
#73425=CARTESIAN_POINT ( 'NONE',  ( 19.14369761974795026, -288.8696336920671683, -221.2751905687686076 ) ) ;
#73426=CARTESIAN_POINT ( 'NONE',  ( -39.22890033885708760, -275.0757377513016877, -345.1706555108469274 ) ) ;
#73427=CARTESIAN_POINT ( 'NONE',  ( 10.60994894321324722, -278.3037151711751562, -327.2992734350243040 ) ) ;
#73428=CARTESIAN_POINT ( 'NONE',  ( 19.04756446975046558, -292.3109305843573793, -318.9764817589377799 ) ) ;
#73429=CARTESIAN_POINT ( 'NONE',  ( -5.485255548961519345, -282.3271771657813929, -201.6190462730926356 ) ) ;
#73431=CARTESIAN_POINT ( 'NONE',  ( -65.32772441722129031, -283.0950140890378179, -337.8200315357108821 ) ) ;
#73432=CARTESIAN_POINT ( 'NONE',  ( -67.25462164755556671, -280.7486541067718235, -199.7444794584705221 ) ) ;
#73433=CARTESIAN_POINT ( 'NONE',  ( -41.56268591078386976, -281.8989929906176712, -346.8997220366821921 ) ) ;
#73434=CARTESIAN_POINT ( 'NONE',  ( -75.20966505104998134, -278.4853843282359094, -337.1356449046780313 ) ) ;
#73435=CARTESIAN_POINT ( 'NONE',  ( 37.80589588287897840, -276.9041209737049485, -257.0371625668553861 ) ) ;
#73436=CARTESIAN_POINT ( 'NONE',  ( -67.74223827176244583, -294.1233781216987495, -207.3071070584150277 ) ) ;
#73439=CARTESIAN_POINT ( 'NONE',  ( -34.40682779664140156, -300.0890474781463695, -195.3601086761975694 ) ) ;
#73440=CARTESIAN_POINT ( 'NONE',  ( -99.98284324329208061, -292.1540947248088855, -232.2781393385183151 ) ) ;
#73441=CARTESIAN_POINT ( 'NONE',  ( -110.3792720864273633, -276.3735023082539897, -285.7676065126699996 ) ) ;
#73442=CARTESIAN_POINT ( 'NONE',  ( -36.08087592867278204, -290.7967163796010368, -346.3502645340448112 ) ) ;
#73443=CARTESIAN_POINT ( 'NONE',  ( -3.581817595367476681, -291.8587435186494190, -205.5216007122476753 ) ) ;
#73444=CARTESIAN_POINT ( 'NONE',  ( 36.32465863657765226, -287.3391725553485117, -292.6058381088807892 ) ) ;
#73446=CARTESIAN_POINT ( 'NONE',  ( -59.20435553746454360, -281.7396051465143501, -340.9021842449895416 ) ) ;
#73447=CARTESIAN_POINT ( 'NONE',  ( -108.5873245166162349, -292.6844130281626235, -249.4610397006937603 ) ) ;
#73448=CARTESIAN_POINT ( 'NONE',  ( -86.17121053890492988, -283.8405413143464671, -215.0988489160258155 ) ) ;
#73449=CARTESIAN_POINT ( 'NONE',  ( -11.58590916279530703, -281.7097850003869439, -201.4750256364088443 ) ) ;
#73450=CARTESIAN_POINT ( 'NONE',  ( -113.5784071327790343, -291.3751527329149553, -279.7873126814164948 ) ) ;
#73451=CARTESIAN_POINT ( 'NONE',  ( -51.84570523314351220, -280.3540118765736224, -198.7019253458057051 ) ) ;
#73452=CARTESIAN_POINT ( 'NONE',  ( -8.645651679697062164, -291.2143832910740571, -199.3361539045705513 ) ) ;
#73453=CARTESIAN_POINT ( 'NONE',  ( 36.53312885592200132, -288.0873470717408509, -249.0377479990441714 ) ) ;
#73454=CARTESIAN_POINT ( 'NONE',  ( 21.44605856236776376, -288.7136953007625380, -319.9950411762073941 ) ) ;
#73455=CARTESIAN_POINT ( 'NONE',  ( -74.72193200695829773, -285.7061762645743670, -207.6577028508007743 ) ) ;
#73457=CARTESIAN_POINT ( 'NONE',  ( 114.7448031289451222, -299.5541904835127980, -197.6977456432065310 ) ) ;
#73458=CARTESIAN_POINT ( 'NONE',  ( 37.62610360218568673, -295.2687894611797219, -259.0492851422251874 ) ) ;
#73459=CARTESIAN_POINT ( 'NONE',  ( -30.65086897587644188, -293.6540545197654524, -346.5748375549480329 ) ) ;
#73460=CARTESIAN_POINT ( 'NONE',  ( -9.911321497236944111, -275.7436910945341424, -338.2789439992577627 ) ) ;
#73461=CARTESIAN_POINT ( 'NONE',  ( -37.24537723390663047, -297.4019209128863395, -193.4622977766161966 ) ) ;
#73462=CARTESIAN_POINT ( 'NONE',  ( 33.00291762288243547, -292.3203290233193457, -292.3234153618646474 ) ) ;
#73463=CARTESIAN_POINT ( 'NONE',  ( -111.2547852393867913, -294.7418986956548110, -274.2120737867838329 ) ) ;
#73464=CARTESIAN_POINT ( 'NONE',  ( 21.30185987935800185, -294.1407577732709910, -226.2242470523301279 ) ) ;
#73465=CARTESIAN_POINT ( 'NONE',  ( 20.77664008092435566, -295.2582137918780631, -315.0637147690405868 ) ) ;
#73467=CARTESIAN_POINT ( 'NONE',  ( -67.51421412072745909, -293.4468762690883068, -339.2062182335864122 ) ) ;
#73468=CARTESIAN_POINT ( 'NONE',  ( -52.23673056871682974, -299.8617427440566985, -196.8027610985576530 ) ) ;
#73469=CARTESIAN_POINT ( 'NONE',  ( -63.89506220021108618, -290.3482339748051686, -338.6674144032093636 ) ) ;
#73470=CARTESIAN_POINT ( 'NONE',  ( -7.975911204908399554, -294.9898209940682250, -337.2307983939592759 ) ) ;
#73471=CARTESIAN_POINT ( 'NONE',  ( -95.56306570372231590, -281.1888393503309658, -222.5009010000722469 ) ) ;
#73472=CARTESIAN_POINT ( 'NONE',  ( -77.22107345109070309, -278.2145518185436117, -205.0086478154535143 ) ) ;
#73474=CARTESIAN_POINT ( 'NONE',  ( -29.84056299386756450, -273.4933441729980359, -193.8297797727026648 ) ) ;
#73475=CARTESIAN_POINT ( 'NONE',  ( 20.81607630902843198, -278.9882978791437154, -223.8962146469456513 ) ) ;
#73476=CARTESIAN_POINT ( 'NONE',  ( -110.5628192823497500, -277.2193277152295536, -249.2635321963098249 ) ) ;
#73477=CARTESIAN_POINT ( 'NONE',  ( -101.8254075753430072, -277.0691194804316524, -231.6351083500380241 ) ) ;
#73479=CARTESIAN_POINT ( 'NONE',  ( -108.5052338887173562, -271.3746457240353607, -251.4275288122364032 ) ) ;
#73482=CARTESIAN_POINT ( 'NONE',  ( -85.44330521762415742, -289.4115182660726759, -212.2878472769111511 ) ) ;
#73483=CARTESIAN_POINT ( 'NONE',  ( -111.9945708100198374, -290.7888183149231622, -251.4414009962390821 ) ) ;
#73484=CARTESIAN_POINT ( 'NONE',  ( -13.66470444066770362, -276.3589537348761382, -199.0208887977689756 ) ) ;
#73485=CARTESIAN_POINT ( 'NONE',  ( -95.30835309555229173, -271.2084113262650362, -222.7504172643921265 ) ) ;
#73486=CARTESIAN_POINT ( 'NONE',  ( -52.13216563256072789, -285.0647485861065888, -194.9052455788024929 ) ) ;
#73488=CARTESIAN_POINT ( 'NONE',  ( -63.69339817169549178, -281.3953674949432866, -340.6333399312136976 ) ) ;
#73491=CARTESIAN_POINT ( 'NONE',  ( -36.18455904326116013, -290.8618652277949082, -196.9606216599541142 ) ) ;
#73492=CARTESIAN_POINT ( 'NONE',  ( -46.86016132879224472, -284.0697312434418222, -196.6870396424370142 ) ) ;
#73495=CARTESIAN_POINT ( 'NONE',  ( 18.23696744037549067, -290.8490223206248970, -219.9260807567870586 ) ) ;
#73496=CARTESIAN_POINT ( 'NONE',  ( -91.54168364009143488, -279.4399775163562936, -320.5233721338743749 ) ) ;
#73497=CARTESIAN_POINT ( 'NONE',  ( -92.13892377627445285, -285.0191047458878870, -323.8893628508005236 ) ) ;
#73498=CARTESIAN_POINT ( 'NONE',  ( -73.23877733225960185, -271.6602502115656534, -203.8145117498533239 ) ) ;
#73499=CARTESIAN_POINT ( 'NONE',  ( -44.02437600801533790, -285.9653070484921500, -197.6676392992300180 ) ) ;
#73500=CARTESIAN_POINT ( 'NONE',  ( 24.27704337199864781, -276.4243948019457093, -230.1304659065303042 ) ) ;
#73501=CARTESIAN_POINT ( 'NONE',  ( -74.08555146273253911, -278.3567728226007034, -333.6263621230654053 ) ) ;
#73502=EDGE_CURVE ( 'NONE', #21957, #66639, #39236, .T. ) ;
#73503=EDGE_CURVE ( 'NONE', #50851, #64529, #75555, .T. ) ;
#73504=CARTESIAN_POINT ( 'NONE',  ( -93.81163797262449577, -285.8669174654083918, -319.7184555395067491 ) ) ;
#73505=ORIENTED_EDGE ( 'NONE', *, *, #58044, .F. ) ;
#73507=CARTESIAN_POINT ( 'NONE',  ( -69.52985433128951342, -295.2975184575709591, -340.3249811405499372 ) ) ;
#73508=CARTESIAN_POINT ( 'NONE',  ( 36.18317175677773889, -289.3621035366091974, -257.1883365611865884 ) ) ;
#73510=CARTESIAN_POINT ( 'NONE',  ( -115.3430155898818299, -275.2662352645559167, -252.5904736702033517 ) ) ;
#73511=CARTESIAN_POINT ( 'NONE',  ( -111.0363889025125133, -277.7397006396163874, -249.1341220442039628 ) ) ;
#73512=CARTESIAN_POINT ( 'NONE',  ( -88.10125266742251426, -289.7554440269162797, -213.5288363139162868 ) ) ;
#73514=CARTESIAN_POINT ( 'NONE',  ( -110.5593206749061608, -285.9572980919892871, -279.1601770277165429 ) ) ;
#73515=CARTESIAN_POINT ( 'NONE',  ( -37.02619628547270025, -281.8162981058169976, -196.3484537016190643 ) ) ;
#73516=CARTESIAN_POINT ( 'NONE',  ( 34.29546097117965076, -288.6387165076610586, -243.7768474168693160 ) ) ;
#73517=CARTESIAN_POINT ( 'NONE',  ( 37.34145334822082418, -283.4568815341990557, -262.9284876403270346 ) ) ;
#73518=CARTESIAN_POINT ( 'NONE',  ( -25.76787376620716330, -277.0752797242349743, -346.4863210879388475 ) ) ;
#73519=CARTESIAN_POINT ( 'NONE',  ( -96.57932617472518189, -295.1973952869595337, -224.9227868701736668 ) ) ;
#73520=CARTESIAN_POINT ( 'NONE',  ( -114.3849361902278190, -278.3699000112984550, -271.6062780342882661 ) ) ;
#73521=CARTESIAN_POINT ( 'NONE',  ( -85.01545242137235903, -299.3089474755935839, -213.1227606144830418 ) ) ;
#73523=CARTESIAN_POINT ( 'NONE',  ( -110.4683760289727132, -293.2662352645559167, -253.7030783399848985 ) ) ;
#73524=CARTESIAN_POINT ( 'NONE',  ( 1.913946225635702492, -272.8097389662971750, -205.2998526814471063 ) ) ;
#73526=CARTESIAN_POINT ( 'NONE',  ( -106.5009479060917243, -278.3744678719471608, -246.6476364827599355 ) ) ;
#73527=CARTESIAN_POINT ( 'NONE',  ( 28.76108799874752364, -277.2636781540074367, -309.0706790704900868 ) ) ;
#73528=CARTESIAN_POINT ( 'NONE',  ( -93.26835507352255661, -282.8908476406718933, -322.9639397607558635 ) ) ;
#73529=CARTESIAN_POINT ( 'NONE',  ( -66.71078729516291617, -291.2022724127160132, -338.3528364119063667 ) ) ;
#73530=CARTESIAN_POINT ( 'NONE',  ( 52.55129206424644650, -300.6784332621725184, -194.0316613479411672 ) ) ;
#73531=CARTESIAN_POINT ( 'NONE',  ( -54.52111395608655897, -299.0412168876722490, -195.7094170107499735 ) ) ;
#73532=CARTESIAN_POINT ( 'NONE',  ( 37.54270597493783868, -295.5572517193583053, -270.7445168673075955 ) ) ;
#73533=CARTESIAN_POINT ( 'NONE',  ( 33.97081688424970736, -279.8473453392966235, -293.2134667184989212 ) ) ;
#73534=CARTESIAN_POINT ( 'NONE',  ( -70.19261666810130862, -271.6372005002476726, -203.3337796091085465 ) ) ;
#73535=CARTESIAN_POINT ( 'NONE',  ( -113.3554383386322684, -286.2284728579659259, -264.3320398969979124 ) ) ;
#73536=CARTESIAN_POINT ( 'NONE',  ( -21.07406231277025199, -287.7587972689769344, -341.8425143912570547 ) ) ;
#73537=CARTESIAN_POINT ( 'NONE',  ( 204.8861687383550816, 294.6280919591721386, -68.62753702822789137 ) ) ;
#73538=EDGE_LOOP ( 'NONE', ( #89326, #26727, #60, #82842 ) ) ;
#73539=CARTESIAN_POINT ( 'NONE',  ( 14.19281757544087696, -286.9201075293059944, -326.8491100629050266 ) ) ;
#73540=CARTESIAN_POINT ( 'NONE',  ( -29.17496981944978529, -288.6125235040371422, -342.9241388872305834 ) ) ;
#73542=CARTESIAN_POINT ( 'NONE',  ( -112.6971453944939014, -285.8141752795130515, -255.8350001204779289 ) ) ;
#73543=CARTESIAN_POINT ( 'NONE',  ( 35.62329281830566430, -275.9375067157598096, -274.3095437789028210 ) ) ;
#73544=CARTESIAN_POINT ( 'NONE',  ( 22.87395351230433960, -291.8345116604801319, -222.8473119626277992 ) ) ;
#73545=CARTESIAN_POINT ( 'NONE',  ( 37.45117085204278595, -282.4280039008593803, -288.2873762213042710 ) ) ;
#73546=CARTESIAN_POINT ( 'NONE',  ( 35.81953328149513993, -283.3488454211931185, -292.2258040050188015 ) ) ;
#73547=CARTESIAN_POINT ( 'NONE',  ( 6.916322366265646338, -282.8014735130303166, -333.4102036834366913 ) ) ;
#73548=CARTESIAN_POINT ( 'NONE',  ( -43.75717589290088227, -280.3022688686673973, -197.5720960716281525 ) ) ;
#73549=CARTESIAN_POINT ( 'NONE',  ( -106.6662871844225293, -275.6237833571633473, -303.7098442033569086 ) ) ;
#73550=CARTESIAN_POINT ( 'NONE',  ( -104.0393943735737139, -256.4255047920307788, -326.8026429627599327 ) ) ;
#73551=EDGE_LOOP ( 'NONE', ( #68319, #2029, #14401, #53030 ) ) ;
#73552=CARTESIAN_POINT ( 'NONE',  ( -32.27152545579270537, -278.9883586153231363, -345.0737192621859890 ) ) ;
#73553=CARTESIAN_POINT ( 'NONE',  ( 24.38510183189676184, -22.52970021484863139, -344.5096856694104872 ) ) ;
#73554=CARTESIAN_POINT ( 'NONE',  ( -64.14634942166337339, -182.0482023548213135, -359.0711594925775216 ) ) ;
#73555=CARTESIAN_POINT ( 'NONE',  ( -110.1510354040710240, -295.9939963101326157, -263.2815451879206989 ) ) ;
#73556=CARTESIAN_POINT ( 'NONE',  ( 38.00292448592740868, -292.8640026154727138, -254.7172259279338391 ) ) ;
#73557=CARTESIAN_POINT ( 'NONE',  ( -93.06201919177942727, -239.3495457806625666, -338.7989358161790392 ) ) ;
#73558=CARTESIAN_POINT ( 'NONE',  ( -98.60903269017077832, -295.7391533980123768, -224.6783599883584657 ) ) ;
#73559=CARTESIAN_POINT ( 'NONE',  ( -85.21934997310023618, -288.1258474033264747, -326.5905929868767998 ) ) ;
#73560=CARTESIAN_POINT ( 'NONE',  ( -28.72955071285097262, -296.8023593552213129, -344.1469527926191745 ) ) ;
#73561=CARTESIAN_POINT ( 'NONE',  ( 23.92983238359569853, -289.4269436513414462, -310.9678868490682930 ) ) ;
#73563=CARTESIAN_POINT ( 'NONE',  ( -44.76091528411387799, -296.0849945215481966, -346.8196975503954604 ) ) ;
#73564=CARTESIAN_POINT ( 'NONE',  ( 16.01512698248800959, -287.3268878716897348, -220.4323636757369513 ) ) ;
#73565=CARTESIAN_POINT ( 'NONE',  ( -80.38913755756647106, -296.2782704323740290, -206.9338987277804449 ) ) ;
#73566=CARTESIAN_POINT ( 'NONE',  ( -79.51435165108738090, -292.3012975219951386, -206.0664719310573787 ) ) ;
#73567=CARTESIAN_POINT ( 'NONE',  ( 29.52429437753199792, -294.5403406068215304, -308.5274708873618579 ) ) ;
#73568=CARTESIAN_POINT ( 'NONE',  ( -46.99656601744062812, -292.0927803124943125, -198.0024034476047348 ) ) ;
#73571=CARTESIAN_POINT ( 'NONE',  ( -34.18823181446925474, -276.0116720405713977, -194.8669470971723285 ) ) ;
#73572=CARTESIAN_POINT ( 'NONE',  ( 9.280884680798010322, -273.4717647087152841, -209.5800082262151420 ) ) ;
#73575=CARTESIAN_POINT ( 'NONE',  ( 18.85397613791859328, -275.7771323264880721, -322.9117875524294732 ) ) ;
#73576=CARTESIAN_POINT ( 'NONE',  ( -35.10209894702379785, -296.5605624607194386, -196.6683717249171366 ) ) ;
#73577=CARTESIAN_POINT ( 'NONE',  ( -51.53994489043085991, -275.3752491977510317, -343.2258922102836323 ) ) ;
#73578=CARTESIAN_POINT ( 'NONE',  ( -110.6508120073928012, -273.6316498264152983, -270.3748327195528987 ) ) ;
#73579=CARTESIAN_POINT ( 'NONE',  ( -76.70074840789855841, -274.4522545458730178, -208.6013109364660068 ) ) ;
#73580=CARTESIAN_POINT ( 'NONE',  ( -91.46325377951568214, -275.0546296546694407, -217.0241566589600097 ) ) ;
#73581=CARTESIAN_POINT ( 'NONE',  ( -82.57225900220493031, -271.4582358020668380, -210.0247447229830584 ) ) ;
#73582=CARTESIAN_POINT ( 'NONE',  ( -86.55248167706605500, -296.4092677367946180, -324.4184176492847200 ) ) ;
#73583=CARTESIAN_POINT ( 'NONE',  ( -31.57413723428266650, -293.5527803757138940, -343.7745020587157683 ) ) ;
#73585=CARTESIAN_POINT ( 'NONE',  ( 26.01977155947634301, -276.6221891280754335, -314.0979365405915473 ) ) ;
#73586=CARTESIAN_POINT ( 'NONE',  ( 26.63550371709898101, -275.2373585112675300, -235.1001529562408621 ) ) ;
#73587=CARTESIAN_POINT ( 'NONE',  ( -112.5105011902911940, -283.4197183812052003, -255.8397595530175295 ) ) ;
#73588=CARTESIAN_POINT ( 'NONE',  ( -112.4783393714420612, -298.5973368360756126, -266.8470104335506221 ) ) ;
#73590=CARTESIAN_POINT ( 'NONE',  ( -60.01899645911787218, -284.9477541320167688, -200.8029268200316153 ) ) ;
#73591=CARTESIAN_POINT ( 'NONE',  ( -104.2768329931730591, -277.2143839710297470, -238.6549452784948642 ) ) ;
#73592=CARTESIAN_POINT ( 'NONE',  ( -54.10565710626204350, -275.8462268937993827, -342.0680240110532964 ) ) ;
#73593=CARTESIAN_POINT ( 'NONE',  ( 22.06278547508822996, -284.1798132737311562, -316.1650495222779682 ) ) ;
#73594=CARTESIAN_POINT ( 'NONE',  ( 34.55660827295164239, -276.9508445634169220, -285.1179386099806266 ) ) ;
#73596=CARTESIAN_POINT ( 'NONE',  ( 31.12740628944732180, -274.3873129190076838, -303.9240512760351294 ) ) ;
#73597=CARTESIAN_POINT ( 'NONE',  ( -76.55828462739536633, -281.5293517990301666, -206.1752872885249985 ) ) ;
#73599=CARTESIAN_POINT ( 'NONE',  ( -80.14302953936375218, -287.3982680931641198, -208.0294958870294408 ) ) ;
#73601=CARTESIAN_POINT ( 'NONE',  ( -111.1587735898196740, -288.3807147593695959, -283.7006271285201819 ) ) ;
#73603=CARTESIAN_POINT ( 'NONE',  ( -87.65882197998212177, -272.0168377754796438, -216.7243889523163602 ) ) ;
#73604=CARTESIAN_POINT ( 'NONE',  ( -110.1548466265458899, -288.5033038766547975, -284.8869173526937857 ) ) ;
#73605=CARTESIAN_POINT ( 'NONE',  ( -89.67076919512652466, -242.4121354169174367, -340.4712336312485377 ) ) ;
#73607=CARTESIAN_POINT ( 'NONE',  ( 38.66592401597007012, -285.9396796532453777, -263.0431830986759110 ) ) ;
#73608=CARTESIAN_POINT ( 'NONE',  ( -5.671344487890855213, -284.2287594886905140, -337.0340707484441509 ) ) ;
#73609=CARTESIAN_POINT ( 'NONE',  ( -103.1514809971601636, -283.2936556743579786, -232.2690778310053474 ) ) ;
#73610=CARTESIAN_POINT ( 'NONE',  ( -103.5563182522245427, -290.9670253668535338, -239.6263762938148716 ) ) ;
#73611=CARTESIAN_POINT ( 'NONE',  ( 34.02258056972365097, -282.7417113555861192, -252.3512885425136574 ) ) ;
#73612=CARTESIAN_POINT ( 'NONE',  ( 35.51213872565642760, -282.2597465318610261, -263.1252304925569661 ) ) ;
#73613=CARTESIAN_POINT ( 'NONE',  ( -29.13079578455961638, -290.9286190153812299, -345.3200292045121387 ) ) ;
#73614=CARTESIAN_POINT ( 'NONE',  ( -106.8259593728122212, -273.3102782501214278, -237.2298335425319920 ) ) ;
#73615=CARTESIAN_POINT ( 'NONE',  ( 22.97762395984459616, -286.2495636713586009, -315.8681871320640084 ) ) ;
#73616=CARTESIAN_POINT ( 'NONE',  ( 32.55306073937912004, -275.1373937609188829, -237.9274532511399229 ) ) ;
#73617=CARTESIAN_POINT ( 'NONE',  ( 0.7266827954646818410, -294.5424129330547203, -206.1532911679029496 ) ) ;
#73620=CARTESIAN_POINT ( 'NONE',  ( -13.38432790028948105, -281.4193779454259356, -339.8937658062558285 ) ) ;
#73621=CARTESIAN_POINT ( 'NONE',  ( -53.75630876482585307, -275.2620294246369781, -343.7669595599688819 ) ) ;
#73623=CARTESIAN_POINT ( 'NONE',  ( -111.8275183238527859, -294.7489197492780022, -286.4329351178544130 ) ) ;
#73624=CARTESIAN_POINT ( 'NONE',  ( 30.27225721122531965, -274.5272212395023530, -242.4388574905363782 ) ) ;
#73625=CARTESIAN_POINT ( 'NONE',  ( -44.38556875275366309, -293.4817096713564979, -196.9538921988186644 ) ) ;
#73626=CARTESIAN_POINT ( 'NONE',  ( -98.50262588172678591, -292.0513734106139623, -229.9856137624763335 ) ) ;
#73627=CARTESIAN_POINT ( 'NONE',  ( -111.3308017882582277, -286.2687808127481048, -273.7059785551666096 ) ) ;
#73629=CARTESIAN_POINT ( 'NONE',  ( 38.02811692269265365, -295.1368341769661470, -283.0101937569141342 ) ) ;
#73630=CARTESIAN_POINT ( 'NONE',  ( 27.62468457497261554, -294.3341909124545737, -229.8547735300761303 ) ) ;
#73631=CARTESIAN_POINT ( 'NONE',  ( -61.01517326468108138, -295.2013572955071936, -339.4695022721770101 ) ) ;
#73632=CARTESIAN_POINT ( 'NONE',  ( 24.41072296049498291, -290.1295099034729787, -312.9471172831084118 ) ) ;
#73633=CARTESIAN_POINT ( 'NONE',  ( -112.2186515861688605, -284.4935601749267562, -288.3736005969368534 ) ) ;
#73634=CARTESIAN_POINT ( 'NONE',  ( -30.61929291252672414, -296.2155323273656791, -194.8032890324896300 ) ) ;
#73635=CARTESIAN_POINT ( 'NONE',  ( -111.8755006756809678, -284.1429300677547189, -289.7450440725257863 ) ) ;
#73636=CARTESIAN_POINT ( 'NONE',  ( -103.2987761474397104, -280.0664363699397654, -305.3112384798483276 ) ) ;
#73638=CARTESIAN_POINT ( 'NONE',  ( -35.91041942542822341, -284.8654224589693058, -196.9780004312582378 ) ) ;
#73639=CARTESIAN_POINT ( 'NONE',  ( 37.64107877718053885, -285.5313494596636588, -268.7537868595474606 ) ) ;
#73640=CARTESIAN_POINT ( 'NONE',  ( -110.1436823427174829, -276.9590822054922796, -249.3807255346758893 ) ) ;
#73642=CARTESIAN_POINT ( 'NONE',  ( -83.68206542277228266, -284.9041392444616463, -213.8103550137312538 ) ) ;
#73643=CARTESIAN_POINT ( 'NONE',  ( 32.03930184909863499, -283.1765404849241463, -302.9559011245347619 ) ) ;
#73644=CARTESIAN_POINT ( 'NONE',  ( -100.4938694101102072, -289.0328068589779491, -314.0031129878314005 ) ) ;
#73645=CARTESIAN_POINT ( 'NONE',  ( -67.37435104295154531, -279.0396481673462858, -340.3931127831607455 ) ) ;
#73646=CARTESIAN_POINT ( 'NONE',  ( -23.01471920588848974, -278.1878725536130332, -345.5683734184902960 ) ) ;
#73647=CARTESIAN_POINT ( 'NONE',  ( -107.9720426774477176, -278.6296312504761090, -251.8633180385693606 ) ) ;
#73648=CARTESIAN_POINT ( 'NONE',  ( -36.74774989060677655, -276.0395415949509470, -195.7059825134823541 ) ) ;
#73649=CARTESIAN_POINT ( 'NONE',  ( 32.18596526420508752, -293.1266176246269310, -237.1478765250244294 ) ) ;
#73650=CARTESIAN_POINT ( 'NONE',  ( 29.86331424860502182, -285.9869643751569015, -303.2778989004222581 ) ) ;
#73651=CARTESIAN_POINT ( 'NONE',  ( -66.72597154568701683, -293.2736642367675586, -200.0546103920527514 ) ) ;
#73652=CARTESIAN_POINT ( 'NONE',  ( -53.22971009541089416, -294.1808874949066421, -341.9800572436694210 ) ) ;
#73653=CARTESIAN_POINT ( 'NONE',  ( -10.48617270934868273, -294.3585642312414734, -338.2644914912154945 ) ) ;
#73654=CARTESIAN_POINT ( 'NONE',  ( -111.6982683039011732, -291.8683150995925644, -251.5307162369283560 ) ) ;
#73655=CARTESIAN_POINT ( 'NONE',  ( 19.75043096694295386, -281.5594486824153933, -224.7060937725205747 ) ) ;
#73656=CARTESIAN_POINT ( 'NONE',  ( -29.08712034845651218, -297.0735580783419323, -193.6716999799625398 ) ) ;
#73657=CARTESIAN_POINT ( 'NONE',  ( 37.27590481853643922, -287.9706976402507053, -251.7727931777235426 ) ) ;
#73658=CARTESIAN_POINT ( 'NONE',  ( 23.25274569757171861, -280.3069879425341355, -315.8431871770719113 ) ) ;
#73659=CARTESIAN_POINT ( 'NONE',  ( 36.36637689983501787, -288.1646676603711512, -292.6074415033127138 ) ) ;
#73660=CARTESIAN_POINT ( 'NONE',  ( 15.04170935009452492, -287.1500975042685013, -219.4880809373403281 ) ) ;
#73661=FACE_OUTER_BOUND ( 'NONE', #56962, .T. ) ;
#73662=CARTESIAN_POINT ( 'NONE',  ( 172.0097273584857476, 242.6675468326081386, -178.1715083274182518 ) ) ;
#73663=CARTESIAN_POINT ( 'NONE',  ( 200.5626873411542022, 290.1978221515497580, -82.34105553867769345 ) ) ;
#73664=CARTESIAN_POINT ( 'NONE',  ( -48.64284848592895827, -276.3967582034913448, -342.6959930051543211 ) ) ;
#73665=CARTESIAN_POINT ( 'NONE',  ( -104.5602964264674597, -277.0792661149073410, -299.7439102515596687 ) ) ;
#73666=CARTESIAN_POINT ( 'NONE',  ( -31.90863132321499052, -297.6261228324871126, -193.4230956962402672 ) ) ;
#73667=CARTESIAN_POINT ( 'NONE',  ( -101.2177587865138122, -255.4137508676264758, -324.7206257864939403 ) ) ;
#73668=CARTESIAN_POINT ( 'NONE',  ( -14.75139343379857237, -275.4503660745291427, -343.5122475340449455 ) ) ;
#73669=CARTESIAN_POINT ( 'NONE',  ( 31.32406147061892554, -295.7362650858349866, -303.0259344471818395 ) ) ;
#73670=CARTESIAN_POINT ( 'NONE',  ( -3.613418446484706781, -293.0023189722448933, -205.5506909153884010 ) ) ;
#73671=CARTESIAN_POINT ( 'NONE',  ( -20.56402232430869859, -299.0600260379783322, -193.5203716029971019 ) ) ;
#73672=CARTESIAN_POINT ( 'NONE',  ( -23.71002232962655043, -287.5592647787937608, -342.6310344664944409 ) ) ;
#73673=CARTESIAN_POINT ( 'NONE',  ( -107.9871450505454078, -273.5924978600625650, -239.8531773425202971 ) ) ;
#73674=CARTESIAN_POINT ( 'NONE',  ( -93.61493184256664790, -297.3782216505862834, -223.8408820521546545 ) ) ;
#73677=CARTESIAN_POINT ( 'NONE',  ( -112.6418127817504882, -280.3848279753441375, -277.2250614057640519 ) ) ;
#73678=CARTESIAN_POINT ( 'NONE',  ( -108.4686597135302435, -279.3979180812686991, -288.1661847545949513 ) ) ;
#73679=CARTESIAN_POINT ( 'NONE',  ( -111.1076879352521161, -280.5440751509220263, -252.0716311130798317 ) ) ;
#73680=CARTESIAN_POINT ( 'NONE',  ( 3.328563963598885955, -273.0891978607116926, -208.8457701666081903 ) ) ;
#73684=CARTESIAN_POINT ( 'NONE',  ( -46.45856240551105287, -280.1000542919696841, -197.8815487093973786 ) ) ;
#73685=CARTESIAN_POINT ( 'NONE',  ( 19.90870854953572788, -275.6577261825014489, -219.0330654206976533 ) ) ;
#73686=CARTESIAN_POINT ( 'NONE',  ( 21.95293194294287176, -278.1820719610389006, -316.3074083321283752 ) ) ;
#73687=CARTESIAN_POINT ( 'NONE',  ( -110.8784302436431943, -276.8647050264839322, -291.1205885337175232 ) ) ;
#73690=CARTESIAN_POINT ( 'NONE',  ( 22.95449566359588189, -284.1466750916733304, -315.5581928751946066 ) ) ;
#73691=CARTESIAN_POINT ( 'NONE',  ( -108.8662801307387298, -289.9518823065682227, -254.9716351141615291 ) ) ;
#73692=CARTESIAN_POINT ( 'NONE',  ( -52.14552365770757092, -285.2161435861906966, -194.8471456306270682 ) ) ;
#73693=CARTESIAN_POINT ( 'NONE',  ( -111.2384876779529321, -282.8568795459104876, -265.3749094065218515 ) ) ;
#73695=CARTESIAN_POINT ( 'NONE',  ( -42.99615841849104214, -281.6995004537365617, -343.7832790167157100 ) ) ;
#73696=CARTESIAN_POINT ( 'NONE',  ( 36.99215484285436872, -285.5693247642517463, -265.5168886629330700 ) ) ;
#73697=CARTESIAN_POINT ( 'NONE',  ( -37.02191670866836404, -281.2613224832580272, -196.9647403827163998 ) ) ;
#73699=CARTESIAN_POINT ( 'NONE',  ( -58.28662483653853599, -281.7181827838107324, -343.6809779964736435 ) ) ;
#73700=CARTESIAN_POINT ( 'NONE',  ( 35.83823662742457117, -295.7639170356713407, -286.8416407754301645 ) ) ;
#73701=CARTESIAN_POINT ( 'NONE',  ( -100.6669930418708674, -278.7022781458733220, -306.9839892094036600 ) ) ;
#73702=CARTESIAN_POINT ( 'NONE',  ( -84.38579946574607504, -287.4065314940246481, -211.7361988700553468 ) ) ;
#73703=CARTESIAN_POINT ( 'NONE',  ( -39.20123149955971797, -293.9491682775845902, -194.8112079111448338 ) ) ;
#73704=CARTESIAN_POINT ( 'NONE',  ( 37.08768832890161349, -273.6758569551037681, -280.0081805225850076 ) ) ;
#73705=CARTESIAN_POINT ( 'NONE',  ( -9.631121957500443642, -287.8963223875177277, -342.0289816169834580 ) ) ;
#73706=CARTESIAN_POINT ( 'NONE',  ( 35.50688522963516647, -291.7968554212936283, -258.4699331130584028 ) ) ;
#73708=CARTESIAN_POINT ( 'NONE',  ( -110.6616344576441691, -277.1617631064543730, -276.1008324570767059 ) ) ;
#73709=CARTESIAN_POINT ( 'NONE',  ( -107.1568040914610549, -294.3594249170555486, -295.7456499766643105 ) ) ;
#73710=CARTESIAN_POINT ( 'NONE',  ( -73.77498017898039961, -290.8618641948971799, -334.2024188173149355 ) ) ;
#73713=CARTESIAN_POINT ( 'NONE',  ( 38.75113981520446060, -291.9599899316522738, -264.6525752021095172 ) ) ;
#73714=CARTESIAN_POINT ( 'NONE',  ( 5.169741830558485240, -288.2375378929597218, -209.9726644693475350 ) ) ;
#73715=CARTESIAN_POINT ( 'NONE',  ( -113.3545673421658648, -288.8173870666251446, -268.3587500776523029 ) ) ;
#73716=CARTESIAN_POINT ( 'NONE',  ( 28.17452688350138601, -288.5244254239260613, -236.7376439021539056 ) ) ;
#73717=DIRECTION ( 'NONE',  ( -1.000000000000000000, -0.000000000000000000, -0.000000000000000000 ) ) ;
#73718=CARTESIAN_POINT ( 'NONE',  ( 34.72465733445011438, -288.1852340720965913, -257.4643935687864769 ) ) ;
#73719=CARTESIAN_POINT ( 'NONE',  ( -2.700661915091799870, -296.5762869281131202, -337.2820061819716670 ) ) ;
#73721=CARTESIAN_POINT ( 'NONE',  ( -4.489367707384485762, -289.8339165161353321, -339.5761962308149009 ) ) ;
#73722=CARTESIAN_POINT ( 'NONE',  ( -97.25298841204069333, -277.1951343289675265, -224.6340422650594348 ) ) ;
#73723=CARTESIAN_POINT ( 'NONE',  ( -113.2163645477496061, -279.0479534217701030, -257.3695980268642529 ) ) ;
#73724=CARTESIAN_POINT ( 'NONE',  ( -72.49337008041595709, -279.2664867021431405, -201.8621341704333929 ) ) ;
#73725=CARTESIAN_POINT ( 'NONE',  ( -63.22995514473932133, -283.7149093591689279, -199.9154083422040458 ) ) ;
#73726=DIRECTION ( 'NONE',  ( -1.000000000000000000, -0.000000000000000000, -0.000000000000000000 ) ) ;
#73727=CARTESIAN_POINT ( 'NONE',  ( -11.28780985351950861, -278.5347071759974256, -200.7937257455134556 ) ) ;
#73728=CARTESIAN_POINT ( 'NONE',  ( -73.33904704047141365, -281.5290120307544157, -336.2156664521891116 ) ) ;
#73729=CARTESIAN_POINT ( 'NONE',  ( -104.9195950068973247, -260.6502555361738018, -315.6180979797861141 ) ) ;
#73730=CARTESIAN_POINT ( 'NONE',  ( -95.63219835742853547, -276.3624001833008492, -319.6248253433047921 ) ) ;
#73731=CARTESIAN_POINT ( 'NONE',  ( -65.85872123725167171, -299.1922791858725645, -202.4090226470799792 ) ) ;
#73732=CARTESIAN_POINT ( 'NONE',  ( -83.70730369116959935, -282.5917432765307922, -331.5156693667757963 ) ) ;
#73733=CARTESIAN_POINT ( 'NONE',  ( -109.7440779004766256, -273.4979115589378011, -259.5027959293468030 ) ) ;
#73734=CARTESIAN_POINT ( 'NONE',  ( -91.76224254228044686, -274.7198147158087522, -216.7233434610150482 ) ) ;
#73735=CARTESIAN_POINT ( 'NONE',  ( 29.10704942818989593, -274.8093255014956640, -239.9625370447037938 ) ) ;
#73736=CARTESIAN_POINT ( 'NONE',  ( -17.67210618421144019, -296.7985928854120630, -342.7358906590718561 ) ) ;
#73737=CARTESIAN_POINT ( 'NONE',  ( -103.7973530481297075, -290.2114433359136001, -309.3593278020074990 ) ) ;
#73738=CARTESIAN_POINT ( 'NONE',  ( -64.20703467292696587, -277.7843467449993682, -199.6832325289846892 ) ) ;
#73739=CARTESIAN_POINT ( 'NONE',  ( -111.5425395019756252, -290.1277284527902793, -290.9338047475022222 ) ) ;
#73740=CARTESIAN_POINT ( 'NONE',  ( -97.54915770768187144, -289.0315988377550411, -312.0781245275720721 ) ) ;
#73741=CARTESIAN_POINT ( 'NONE',  ( 17.95866809632716254, -290.8443932923930788, -219.6968315096645483 ) ) ;
#73744=CARTESIAN_POINT ( 'NONE',  ( -105.7660700396458822, -290.4029477440144547, -244.6032623194039672 ) ) ;
#73746=CARTESIAN_POINT ( 'NONE',  ( -52.13970387330772382, -286.8085524760460316, -194.9820007753183120 ) ) ;
#73747=CARTESIAN_POINT ( 'NONE',  ( 30.91033621190086578, -290.2662352645559167, -285.9065529553535612 ) ) ;
#73748=CARTESIAN_POINT ( 'NONE',  ( -66.84512178793866610, -294.4881553351906973, -341.2439469251428932 ) ) ;
#73749=CARTESIAN_POINT ( 'NONE',  ( 36.01070059573344651, -283.1439305523996381, -292.2857158972446996 ) ) ;
#73750=CARTESIAN_POINT ( 'NONE',  ( -49.41943863945510174, -285.7273382127859804, -198.3156738816327902 ) ) ;
#73751=CARTESIAN_POINT ( 'NONE',  ( 34.65100332138116812, -277.0609250344158454, -285.1358981638676937 ) ) ;
#73752=CARTESIAN_POINT ( 'NONE',  ( -37.52933173917555365, -290.0699379404213119, -195.7038249997779644 ) ) ;
#73753=CARTESIAN_POINT ( 'NONE',  ( -54.28840429534911038, -272.6245083723702010, -198.9472557324415050 ) ) ;
#73754=ORIENTED_EDGE ( 'NONE', *, *, #82664, .T. ) ;
#73756=CARTESIAN_POINT ( 'NONE',  ( 25.69489922945507843, -293.8035364451362170, -314.5670523385749107 ) ) ;
#73757=CARTESIAN_POINT ( 'NONE',  ( -73.08654553314303826, -287.4947045784555826, -205.0502160175830682 ) ) ;
#73758=CARTESIAN_POINT ( 'NONE',  ( -106.8802828879418172, -297.2162379984434892, -302.7011553453286865 ) ) ;
#73759=CARTESIAN_POINT ( 'NONE',  ( 26.45228736770980049, -287.7147263547475404, -234.5613535756960459 ) ) ;
#73760=CARTESIAN_POINT ( 'NONE',  ( -111.1078145051525894, -277.8780976944817667, -249.1153988151750127 ) ) ;
#73761=CARTESIAN_POINT ( 'NONE',  ( -33.55269532271341859, -292.7500827522039231, -193.5564551725889260 ) ) ;
#73762=CARTESIAN_POINT ( 'NONE',  ( 36.61397865747861147, -285.9016788278399304, -286.8781827619521323 ) ) ;
#73763=CARTESIAN_POINT ( 'NONE',  ( -24.90704448006370697, -295.2311137609514162, -346.3830811067127797 ) ) ;
#73764=CARTESIAN_POINT ( 'NONE',  ( -55.02158141227934607, -292.1517460690146208, -199.5126226953891830 ) ) ;
#73766=FACE_OUTER_BOUND ( 'NONE', #70957, .T. ) ;
#73767=CARTESIAN_POINT ( 'NONE',  ( -101.6167628974910002, -254.6067659492929351, -324.2419241925472875 ) ) ;
#73768=CARTESIAN_POINT ( 'NONE',  ( 29.51467527819651337, -288.5903127428882158, -233.4692965923466659 ) ) ;
#73769=CARTESIAN_POINT ( 'NONE',  ( -2.659677404128736544, -280.1237833571632336, -342.4524372437778652 ) ) ;
#73771=CARTESIAN_POINT ( 'NONE',  ( -103.2967528793522263, -283.0396799742412099, -302.4802008733856269 ) ) ;
#73772=CARTESIAN_POINT ( 'NONE',  ( 22.78724498022210909, -282.9427202189310151, -225.7914021569596628 ) ) ;
#73773=CARTESIAN_POINT ( 'NONE',  ( -101.6854563161719227, -256.6257814484651476, -325.9156231221182338 ) ) ;
#73774=CARTESIAN_POINT ( 'NONE',  ( -100.9388859079359406, -282.5640546632850487, -312.8117763095281703 ) ) ;
#73775=CARTESIAN_POINT ( 'NONE',  ( -11.42785105332955098, -284.4115164783612499, -200.3588378163500181 ) ) ;
#73776=CARTESIAN_POINT ( 'NONE',  ( -8.188134955983059626, -276.2901658752921321, -200.3742206346934154 ) ) ;
#73777=CARTESIAN_POINT ( 'NONE',  ( -95.34174379319205173, -297.6692346955820199, -225.9111981844087040 ) ) ;
#73778=CARTESIAN_POINT ( 'NONE',  ( 20.90386569182295418, -292.8637558888753460, -315.2002126159817976 ) ) ;
#73779=CARTESIAN_POINT ( 'NONE',  ( -112.6194715577560146, -279.4009956492743640, -254.5950386476127392 ) ) ;
#73780=CARTESIAN_POINT ( 'NONE',  ( 16.53115478250300896, -276.2589932042342298, -319.6414663191355885 ) ) ;
#73781=CARTESIAN_POINT ( 'NONE',  ( 19.16138736105685325, -299.6846001230114211, -193.5876150138238074 ) ) ;
#73782=CARTESIAN_POINT ( 'NONE',  ( -17.45137186351961489, -275.7216532141115408, -344.4277592622011639 ) ) ;
#73783=CARTESIAN_POINT ( 'NONE',  ( -114.0438014765299215, -273.4268578961535354, -284.1485094271325806 ) ) ;
#73784=CARTESIAN_POINT ( 'NONE',  ( 35.38724277842326416, -273.3161052442963523, -251.9927585438613278 ) ) ;
#73785=CARTESIAN_POINT ( 'NONE',  ( -70.53536832136332180, -296.9064252494713969, -339.1998332857435230 ) ) ;
#73786=DIRECTION ( 'NONE',  ( -1.000000000000000000, -0.000000000000000000, -0.000000000000000000 ) ) ;
#73788=CARTESIAN_POINT ( 'NONE',  ( -64.15568773085546184, -284.4900749232543262, -338.5904089261549643 ) ) ;
#73789=CARTESIAN_POINT ( 'NONE',  ( -91.69306513445995677, -285.5740807330581106, -323.4638781271057155 ) ) ;
#73790=CARTESIAN_POINT ( 'NONE',  ( -22.43094972540467325, -285.5965859655285612, -198.7440730104717659 ) ) ;
#73791=CARTESIAN_POINT ( 'NONE',  ( -107.8873185852755370, -276.6660275418012134, -292.2062575061756888 ) ) ;
#73792=CARTESIAN_POINT ( 'NONE',  ( -106.7277233849747375, -286.7590490024441578, -243.9708687387712587 ) ) ;
#73793=CARTESIAN_POINT ( 'NONE',  ( -22.03164190960058377, -278.7315944653297493, -198.2233311138994907 ) ) ;
#73795=CARTESIAN_POINT ( 'NONE',  ( 25.64816641636719652, -277.1452475668247075, -307.8644883084474486 ) ) ;
#73798=CARTESIAN_POINT ( 'NONE',  ( -90.24548739326772306, -273.7707272385108581, -219.9525582034610807 ) ) ;
#73799=CARTESIAN_POINT ( 'NONE',  ( 35.45939109536712408, -282.6670921712283189, -295.1062011347452767 ) ) ;
#73800=CARTESIAN_POINT ( 'NONE',  ( -38.72514932449956149, -283.5614130177448828, -347.2871407044924013 ) ) ;
#73804=CARTESIAN_POINT ( 'NONE',  ( 19.34654445579052862, -288.7197857380605797, -220.0169296502561167 ) ) ;
#73805=CARTESIAN_POINT ( 'NONE',  ( -109.4332341122041754, -295.9134067552732290, -257.8946647959382972 ) ) ;
#73806=CARTESIAN_POINT ( 'NONE',  ( -0.8449143339587453783, -291.8724508696616908, -202.6758358785880034 ) ) ;
#73807=CARTESIAN_POINT ( 'NONE',  ( -13.07767898527680295, -287.2109539346897691, -339.9453477319760282 ) ) ;
#73808=CARTESIAN_POINT ( 'NONE',  ( -18.33870979613791619, -287.3773197666213832, -341.5074526759464675 ) ) ;
#73810=CARTESIAN_POINT ( 'NONE',  ( 16.25398396665944745, -288.0395014047340396, -220.1964574321729629 ) ) ;
#73811=CARTESIAN_POINT ( 'NONE',  ( -112.0492067503147382, -276.6442006755905823, -263.1794260992977001 ) ) ;
#73812=CARTESIAN_POINT ( 'NONE',  ( -45.95578702752110445, -287.5593842692071576, -346.1252375044198288 ) ) ;
#73813=CARTESIAN_POINT ( 'NONE',  ( 14.88766819689077003, -288.7885883979220694, -216.5364607004050868 ) ) ;
#73814=CARTESIAN_POINT ( 'NONE',  ( -29.20164869531769369, -286.9492078427433057, -345.1379825956768173 ) ) ;
#73815=CARTESIAN_POINT ( 'NONE',  ( -26.69676767428009967, -283.8548206379275030, -342.8701154712414905 ) ) ;
#73816=CARTESIAN_POINT ( 'NONE',  ( -95.18478502880068959, -293.2136646698784830, -222.3390730214786117 ) ) ;
#73817=CARTESIAN_POINT ( 'NONE',  ( 82.14122032850023913, -300.1543061692601668, -193.4499960878401623 ) ) ;
#73819=CARTESIAN_POINT ( 'NONE',  ( -111.7808693500708159, -298.3032906383199929, -283.6225164144282189 ) ) ;
#73820=CARTESIAN_POINT ( 'NONE',  ( -14.24823353745979482, -279.5564611225354952, -200.8864260453578652 ) ) ;
#73821=CARTESIAN_POINT ( 'NONE',  ( 37.12240448217178113, -279.6723202601086768, -279.7327463155705800 ) ) ;
#73822=CARTESIAN_POINT ( 'NONE',  ( -41.94612645753468172, -294.3058208084767102, -347.1138451097400548 ) ) ;
#73823=CARTESIAN_POINT ( 'NONE',  ( -110.5822304238010503, -270.9353513147710828, -259.3439437264424328 ) ) ;
#73824=CARTESIAN_POINT ( 'NONE',  ( -35.09826129485670521, -275.1036056119682485, -344.7673084690574115 ) ) ;
#73825=CARTESIAN_POINT ( 'NONE',  ( -26.11566802437828017, -296.2214099567489711, -342.9918255394018729 ) ) ;
#73827=CARTESIAN_POINT ( 'NONE',  ( -67.28786665653916543, -272.2417987862393716, -200.0629430128183799 ) ) ;
#73828=CARTESIAN_POINT ( 'NONE',  ( -83.58649898465269246, -293.9161297838734299, -330.7216908243435682 ) ) ;
#73829=CARTESIAN_POINT ( 'NONE',  ( 28.93305158235684615, -295.4081990845666610, -302.4635687803697124 ) ) ;
#73830=CARTESIAN_POINT ( 'NONE',  ( -4.254505052825189537, -295.4072536823830433, -335.6272686060038950 ) ) ;
#73832=CARTESIAN_POINT ( 'NONE',  ( -37.94346067913136267, -284.0647605629362147, -195.0083164981553523 ) ) ;
#73833=CARTESIAN_POINT ( 'NONE',  ( -98.73330315598403217, -296.0044225332788415, -309.9514553950112372 ) ) ;
#73834=CARTESIAN_POINT ( 'NONE',  ( -112.3597286615845974, -284.7692380986950980, -253.0032553564617785 ) ) ;
#73835=CARTESIAN_POINT ( 'NONE',  ( 33.96054671114661971, -283.1490896012176677, -245.1989188759397393 ) ) ;
#73836=CARTESIAN_POINT ( 'NONE',  ( -102.4983191144708741, -284.7558070208886534, -229.3689322181430441 ) ) ;
#73837=CARTESIAN_POINT ( 'NONE',  ( -111.0789092493111099, -288.7200106634448957, -257.3044641378569395 ) ) ;
#73838=CARTESIAN_POINT ( 'NONE',  ( -4.771743288812454686, -271.9809262143061233, -202.8022627189028810 ) ) ;
#73839=CARTESIAN_POINT ( 'NONE',  ( -72.59595684809394811, -284.2598991290782919, -205.8612979581295690 ) ) ;
#73840=CARTESIAN_POINT ( 'NONE',  ( -112.2663082739289564, -289.2670012222915830, -286.7255796422575145 ) ) ;
#73842=CARTESIAN_POINT ( 'NONE',  ( -111.5982237241403823, -279.7496748086906564, -288.4318337455994197 ) ) ;
#73843=CARTESIAN_POINT ( 'NONE',  ( -19.69740637617231016, -292.8466233125772078, -343.6752236016824895 ) ) ;
#73844=CARTESIAN_POINT ( 'NONE',  ( 19.69519086606120695, -280.5749137806306521, -224.7663753842709866 ) ) ;
#73845=CARTESIAN_POINT ( 'NONE',  ( -47.62947259828213475, -295.3461899170790730, -346.6707618167072837 ) ) ;
#73846=CARTESIAN_POINT ( 'NONE',  ( -84.59301588795722182, -283.4868478609280942, -211.3981859481368701 ) ) ;
#73847=CARTESIAN_POINT ( 'NONE',  ( -89.68118424490572238, -281.3146599581779697, -216.5711059396477651 ) ) ;
#73848=CARTESIAN_POINT ( 'NONE',  ( -69.83922304417063742, -294.5497814741926277, -335.9912898032399085 ) ) ;
#73849=CARTESIAN_POINT ( 'NONE',  ( -86.81020433254104773, -271.3662507241008939, -213.6978074929134834 ) ) ;
#73852=CARTESIAN_POINT ( 'NONE',  ( 26.98908576708132401, -284.0417792222714297, -308.3235406939451195 ) ) ;
#73853=CARTESIAN_POINT ( 'NONE',  ( -39.69729818416332989, -294.5901478204166324, -343.3971139300035702 ) ) ;
#73855=CARTESIAN_POINT ( 'NONE',  ( -95.99890600148557951, -275.4094976428775681, -317.0979686699210447 ) ) ;
#73856=CARTESIAN_POINT ( 'NONE',  ( -38.34502749961526291, -273.2370464740843659, -193.5291444596736028 ) ) ;
#73857=CARTESIAN_POINT ( 'NONE',  ( -103.5554268108481324, -290.8003721497686911, -239.6244557814866027 ) ) ;
#73858=CARTESIAN_POINT ( 'NONE',  ( -96.17687782110718331, -280.6899571714385502, -225.9652891420465153 ) ) ;
#73859=CARTESIAN_POINT ( 'NONE',  ( -95.25302026304424885, -274.7907954267257082, -224.6148676669409667 ) ) ;
#73860=CARTESIAN_POINT ( 'NONE',  ( -1.987035912855077413, -284.1919728182602398, -337.8628819255183089 ) ) ;
#73861=CARTESIAN_POINT ( 'NONE',  ( -19.42284112748631131, -279.0826062357957085, -199.1323857647484203 ) ) ;
#73862=CARTESIAN_POINT ( 'NONE',  ( 22.44627944024040644, -278.1716316236181683, -315.6424403049408625 ) ) ;
#73864=CARTESIAN_POINT ( 'NONE',  ( -88.03477456345915186, -273.1994360773490484, -212.3315192770881197 ) ) ;
#73865=CARTESIAN_POINT ( 'NONE',  ( -27.94840955108134750, -294.0923447998343931, -196.4643949375640659 ) ) ;
#73868=CARTESIAN_POINT ( 'NONE',  ( -39.10325494934452450, -293.2136277450637181, -346.1054405960279610 ) ) ;
#73870=CARTESIAN_POINT ( 'NONE',  ( -55.29475553308035529, -297.4816189100373549, -199.5290269991330945 ) ) ;
#73872=CARTESIAN_POINT ( 'NONE',  ( -7.479538313361029367, -293.9567322257258866, -200.1261392262484264 ) ) ;
#73873=CARTESIAN_POINT ( 'NONE',  ( 108.5619616845123971, -302.2645883696979467, -190.3030568020281805 ) ) ;
#73874=CARTESIAN_POINT ( 'NONE',  ( -6.278151174005602186, -288.4613230929442125, -202.2655952638983194 ) ) ;
#73875=CARTESIAN_POINT ( 'NONE',  ( -41.99542039640643054, -275.1107534586386123, -345.0625258940852405 ) ) ;
#73876=CARTESIAN_POINT ( 'NONE',  ( 37.04214408809731651, -277.5241241732517210, -274.3661998222550551 ) ) ;
#73877=CARTESIAN_POINT ( 'NONE',  ( 11.21264757630517295, -292.4531601628782482, -326.7861967517209791 ) ) ;
#73878=CARTESIAN_POINT ( 'NONE',  ( -66.90272753528901717, -281.5292724995988465, -200.6011642793420719 ) ) ;
#73879=ORIENTED_EDGE ( 'NONE', *, *, #77244, .F. ) ;
#73880=CARTESIAN_POINT ( 'NONE',  ( -64.06706087006881489, -283.0773503888726736, -338.3158277531293834 ) ) ;
#73881=CARTESIAN_POINT ( 'NONE',  ( -75.17170661637928220, -278.6237813932754079, -337.0723098398895559 ) ) ;
#73882=CARTESIAN_POINT ( 'NONE',  ( -1.831900275020204472, -281.3872222048400431, -338.2364657459490900 ) ) ;
#73883=CARTESIAN_POINT ( 'NONE',  ( -34.28841866488321699, -277.9558883237970690, -347.0650793260665523 ) ) ;
#73885=CARTESIAN_POINT ( 'NONE',  ( 23.82360943416126986, -277.6846734358366007, -315.9847156104772807 ) ) ;
#73886=CARTESIAN_POINT ( 'NONE',  ( -6.998514795304313196, -294.9805209788416391, -207.2794874003663779 ) ) ;
#73888=CARTESIAN_POINT ( 'NONE',  ( -106.6190931217805087, -298.9273471183138895, -241.6271056257840257 ) ) ;
#73889=CARTESIAN_POINT ( 'NONE',  ( -88.15471438379844926, -292.4004734663049021, -217.4490762572561096 ) ) ;
#73890=CARTESIAN_POINT ( 'NONE',  ( -41.98350225846543538, -275.1310184801379819, -344.8743369305223041 ) ) ;
#73891=CARTESIAN_POINT ( 'NONE',  ( -92.83719101655950112, -291.5942743863346891, -322.3428438578150690 ) ) ;
#73892=CARTESIAN_POINT ( 'NONE',  ( -92.62815983957735000, -290.5812807393708681, -222.5353922588550688 ) ) ;
#73893=CARTESIAN_POINT ( 'NONE',  ( 20.52247575971392735, -287.7465773972697320, -321.0885967068805371 ) ) ;
#73895=CARTESIAN_POINT ( 'NONE',  ( -109.1391143042689436, -283.1754909391347610, -253.2312859296519889 ) ) ;
#73896=CARTESIAN_POINT ( 'NONE',  ( -69.26809409742949697, -291.3371681885150792, -337.3803006998751925 ) ) ;
#73897=CARTESIAN_POINT ( 'NONE',  ( -79.69205875168110254, -283.9483635898707234, -209.9896532683062560 ) ) ;
#73899=CARTESIAN_POINT ( 'NONE',  ( 21.71533229932875386, -282.2578444688995205, -226.5962534668126978 ) ) ;
#73900=CARTESIAN_POINT ( 'NONE',  ( -51.62972456036622759, -290.1718923654533455, -345.7844072912005799 ) ) ;
#73901=CARTESIAN_POINT ( 'NONE',  ( -69.77325112503888249, -280.1055240545388187, -204.8783137650117396 ) ) ;
#73902=CARTESIAN_POINT ( 'NONE',  ( -64.23495259808915137, -290.5039918610806353, -198.5782455056484821 ) ) ;
#73903=CARTESIAN_POINT ( 'NONE',  ( 9.703807935584841005, -287.4840925372035940, -209.6085131739653775 ) ) ;
#73904=CARTESIAN_POINT ( 'NONE',  ( 30.07461289773250712, -287.5627034143271317, -233.1754279496403797 ) ) ;
#73905=CARTESIAN_POINT ( 'NONE',  ( -35.93559594995342366, -286.2369562790522650, -197.3746611869852927 ) ) ;
#73908=CARTESIAN_POINT ( 'NONE',  ( 23.80336376861723835, -294.8088618346456542, -225.6220227360954027 ) ) ;
#73909=CARTESIAN_POINT ( 'NONE',  ( -101.2257768192920082, -294.6788166068431565, -312.5535512445609925 ) ) ;
#73910=CARTESIAN_POINT ( 'NONE',  ( -6.187383634769226148, -275.6911965959109239, -336.6532594284458924 ) ) ;
#73911=CARTESIAN_POINT ( 'NONE',  ( -35.82231046780808725, -297.4192976348145407, -193.4632129206172237 ) ) ;
#73912=CARTESIAN_POINT ( 'NONE',  ( 23.92835671900255790, -291.4687502070530059, -229.4137384997679590 ) ) ;
#73913=CARTESIAN_POINT ( 'NONE',  ( -101.0499860729498778, -294.2802809457257354, -308.1347300222603280 ) ) ;
#73914=CARTESIAN_POINT ( 'NONE',  ( -98.63956921055091698, -292.3151546047912461, -229.8992058195396453 ) ) ;
#73915=CARTESIAN_POINT ( 'NONE',  ( 19.57713208129874971, -293.9806969196148430, -224.1409160332540864 ) ) ;
#73917=CARTESIAN_POINT ( 'NONE',  ( 26.53421145933675263, -292.0839678369325725, -310.0807717358518971 ) ) ;
#73918=CARTESIAN_POINT ( 'NONE',  ( -71.72753629290552624, -299.5979734891082558, -203.6939506260904409 ) ) ;
#73919=CARTESIAN_POINT ( 'NONE',  ( -56.11437692538834199, -290.2410734688080538, -341.2022243196234399 ) ) ;
#73920=CARTESIAN_POINT ( 'NONE',  ( -53.74804602735255799, -279.2414416841962748, -343.9621137417991008 ) ) ;
#73921=CARTESIAN_POINT ( 'NONE',  ( -110.0755937367490418, -277.5393388361014217, -246.4638037918190605 ) ) ;
#73922=CARTESIAN_POINT ( 'NONE',  ( -18.56681917932296599, -273.6362941101798469, -195.7352761255145026 ) ) ;
#73923=CARTESIAN_POINT ( 'NONE',  ( 33.59625934825948690, -279.9273388536918219, -293.0925086881986772 ) ) ;
#73924=CARTESIAN_POINT ( 'NONE',  ( -64.43859120765851856, -278.1043208008236434, -199.0861079120081740 ) ) ;
#73925=CARTESIAN_POINT ( 'NONE',  ( -107.9283820667177736, -295.5058280006942937, -249.8973985858545745 ) ) ;
#73927=CARTESIAN_POINT ( 'NONE',  ( -21.92060251988330677, -274.9064447384953951, -198.9042609540987314 ) ) ;
#73930=CARTESIAN_POINT ( 'NONE',  ( -112.3666653663188839, -288.6691802253907895, -262.7768855651746094 ) ) ;
#73931=CARTESIAN_POINT ( 'NONE',  ( -105.1559689240054212, -290.0805981575247188, -306.8333669901844019 ) ) ;
#73932=CARTESIAN_POINT ( 'NONE',  ( -11.01419554982314075, -276.3945657467878618, -199.9005619880542781 ) ) ;
#73933=CARTESIAN_POINT ( 'NONE',  ( -89.38284643684882269, -295.3175821860816654, -216.5138247584088731 ) ) ;
#73935=CARTESIAN_POINT ( 'NONE',  ( -13.48180273340718571, -281.9471979166174265, -343.4012721203852720 ) ) ;
#73937=CARTESIAN_POINT ( 'NONE',  ( 2.706147341885323243, -280.5152443130122606, -333.8344045608845931 ) ) ;
#73939=CARTESIAN_POINT ( 'NONE',  ( -14.70946362963264065, -291.1470087163989433, -200.5405452603425260 ) ) ;
#73940=CARTESIAN_POINT ( 'NONE',  ( -90.53162389273815336, -283.4288544204246705, -218.5022676429446449 ) ) ;
#73941=FACE_OUTER_BOUND ( 'NONE', #73095, .T. ) ;
#73943=CARTESIAN_POINT ( 'NONE',  ( 0.9515220733797971064, -290.5630023235333397, -205.8736790340005882 ) ) ;
#73944=CARTESIAN_POINT ( 'NONE',  ( -110.6968746167573983, -280.0408341145362670, -278.9024217866071353 ) ) ;
#73945=CARTESIAN_POINT ( 'NONE',  ( -101.0801813714010819, -285.1939784076167257, -312.9464394515257482 ) ) ;
#73946=CARTESIAN_POINT ( 'NONE',  ( -31.34941537011497203, -272.2070926714131929, -195.0260647574129962 ) ) ;
#73947=CARTESIAN_POINT ( 'NONE',  ( -67.54769721631765833, -285.6444702736058616, -203.9036297671191846 ) ) ;
#73948=CARTESIAN_POINT ( 'NONE',  ( -4.789228989113279766, -278.0401137696960063, -336.3729365570699201 ) ) ;
#73949=CARTESIAN_POINT ( 'NONE',  ( 5.499601202870486816, -277.2584797257404716, -329.7298779904547246 ) ) ;
#73950=CARTESIAN_POINT ( 'NONE',  ( -111.6150036585392087, -286.4138848813902314, -281.1422890198280129 ) ) ;
#73953=CARTESIAN_POINT ( 'NONE',  ( -77.08404761448591103, -295.4021818777276849, -336.3742362034354869 ) ) ;
#73954=CARTESIAN_POINT ( 'NONE',  ( 29.11119913181458685, -289.0789560618642327, -236.2493032309313321 ) ) ;
#73956=CARTESIAN_POINT ( 'NONE',  ( -55.63300648810263738, -292.7666405000204577, -350.3538533559490702 ) ) ;
#73957=CARTESIAN_POINT ( 'NONE',  ( -68.53415931668918404, -278.5721433217157141, -200.2859392594817791 ) ) ;
#73958=CARTESIAN_POINT ( 'NONE',  ( -39.17183834611936533, -290.4294551764250514, -194.1701960755857215 ) ) ;
#73960=CARTESIAN_POINT ( 'NONE',  ( -94.67354007227584134, -286.7210794403503655, -224.0402700283262050 ) ) ;
#73961=CARTESIAN_POINT ( 'NONE',  ( -107.4112342350791067, -280.6265932114612838, -246.3659205339392599 ) ) ;
#73962=CARTESIAN_POINT ( 'NONE',  ( 38.38885664596990921, -288.8492132832033690, -260.1881605336885741 ) ) ;
#73963=CARTESIAN_POINT ( 'NONE',  ( 2.176196039675799554, -284.5235453667215211, -334.1660781397623055 ) ) ;
#73964=CARTESIAN_POINT ( 'NONE',  ( 37.23927360239664353, -275.9584694388872776, -289.5099655181301159 ) ) ;
#73965=CARTESIAN_POINT ( 'NONE',  ( -50.21330951316453195, -295.9071516055281563, -196.8344665436037246 ) ) ;
#73966=CARTESIAN_POINT ( 'NONE',  ( -16.98994805964158417, -280.1412381099899562, -196.0993768756424060 ) ) ;
#73967=CARTESIAN_POINT ( 'NONE',  ( -73.56864489035299925, -299.4875645629279575, -205.3309505810239841 ) ) ;
#73970=CARTESIAN_POINT ( 'NONE',  ( -29.91532298040375792, -272.3847949563289603, -194.7382184377183023 ) ) ;
#73972=CARTESIAN_POINT ( 'NONE',  ( -95.32568175659837095, -277.4349709954749414, -314.8116108522064565 ) ) ;
#73973=CARTESIAN_POINT ( 'NONE',  ( -2.750648921129092539, -275.7042312916930769, -201.9983547557986867 ) ) ;
#73974=CARTESIAN_POINT ( 'NONE',  ( 31.81471935147924768, -280.1807685078698000, -236.9189749165308001 ) ) ;
#73975=CARTESIAN_POINT ( 'NONE',  ( -20.88249082309033255, -290.5981528987918523, -342.5211376605471401 ) ) ;
#73976=CARTESIAN_POINT ( 'NONE',  ( -113.5417001291470882, -274.1520230306431358, -270.3814460222293405 ) ) ;
#73977=CARTESIAN_POINT ( 'NONE',  ( -36.20720205948475723, -299.2711283777799736, -193.7579611739544987 ) ) ;
#73978=CARTESIAN_POINT ( 'NONE',  ( -68.58937396217021387, -293.6407473853936949, -202.3498941708393204 ) ) ;
#73979=CARTESIAN_POINT ( 'NONE',  ( 11.07595942897569152, -280.3803540244982742, -327.4884985235727299 ) ) ;
#73980=CARTESIAN_POINT ( 'NONE',  ( 36.78390087520668317, -283.3768880073544665, -262.9848089022532349 ) ) ;
#73981=CARTESIAN_POINT ( 'NONE',  ( -82.03613388021695130, -271.4600018336710150, -210.5112076429528543 ) ) ;
#73982=CARTESIAN_POINT ( 'NONE',  ( -110.9537752465019054, -286.4036669783151865, -250.4724264816589141 ) ) ;
#73983=CARTESIAN_POINT ( 'NONE',  ( 22.20477840730272234, -287.0677375418065367, -313.1214146159805978 ) ) ;
#73984=CARTESIAN_POINT ( 'NONE',  ( 181.4475197844431023, 253.2525738607984636, -166.6027886999133614 ) ) ;
#73986=CARTESIAN_POINT ( 'NONE',  ( -37.51858574207007280, -287.6290242378129847, -346.7846581648530560 ) ) ;
#73987=CARTESIAN_POINT ( 'NONE',  ( -48.06828069080074783, -288.8589574907578594, -342.6411516971366495 ) ) ;
#73988=ORIENTED_EDGE ( 'NONE', *, *, #60912, .T. ) ;
#73989=CARTESIAN_POINT ( 'NONE',  ( -113.8445911960692740, -285.7080996857646937, -264.2864697702846684 ) ) ;
#73990=CARTESIAN_POINT ( 'NONE',  ( 9.495392128865923098, -275.0500366565785271, -214.2737113012912857 ) ) ;
#73991=CARTESIAN_POINT ( 'NONE',  ( 15.23629030490137204, -291.6938436256614295, -214.4576656514300623 ) ) ;
#73992=CARTESIAN_POINT ( 'NONE',  ( -2.931002068478880673, -283.2608556296496545, -339.1450526373840830 ) ) ;
#73994=CARTESIAN_POINT ( 'NONE',  ( 32.53024891969280930, -282.6775741676256075, -239.6916137929241017 ) ) ;
#73995=CARTESIAN_POINT ( 'NONE',  ( 17.81409120262141244, -282.6225527137782478, -324.1362916875922906 ) ) ;
#73997=CARTESIAN_POINT ( 'NONE',  ( 31.98288692825983404, -272.6237833571632905, -237.0123917617631264 ) ) ;
#73998=CARTESIAN_POINT ( 'NONE',  ( -113.5233723423151844, -274.1796448693337425, -270.3818398631209448 ) ) ;
#74000=CARTESIAN_POINT ( 'NONE',  ( 34.66882665568951438, -277.8154144072465215, -290.7676487879307956 ) ) ;
#74001=CARTESIAN_POINT ( 'NONE',  ( 83.75835951168025417, 83.55189833975310876, -301.8609685986378963 ) ) ;
#74002=CARTESIAN_POINT ( 'NONE',  ( -92.81635225106667519, -296.5777067063164623, -222.7345601121778316 ) ) ;
#74003=CARTESIAN_POINT ( 'NONE',  ( 22.16565205169789721, -292.4044017913836342, -221.5922555796551023 ) ) ;
#74004=CARTESIAN_POINT ( 'NONE',  ( -69.44094709307063340, -196.3684237509906438, -356.8806884016171921 ) ) ;
#74005=CARTESIAN_POINT ( 'NONE',  ( -9.360389901375182120, -296.9707284207239582, -193.9569664623705023 ) ) ;
#74006=CARTESIAN_POINT ( 'NONE',  ( -78.63877396349961657, -288.0180704208287352, -331.5863002574434404 ) ) ;
#74007=CARTESIAN_POINT ( 'NONE',  ( -94.01021694886543401, -297.7421531344366485, -318.3343705354888016 ) ) ;
#74008=CARTESIAN_POINT ( 'NONE',  ( 31.43018154816243381, -288.5220917264987293, -244.3009173340606992 ) ) ;
#74010=CARTESIAN_POINT ( 'NONE',  ( 22.99419793529893141, -295.1302093936623123, -317.8416640315668928 ) ) ;
#74011=CARTESIAN_POINT ( 'NONE',  ( -93.46532047161268508, -284.3812961703030169, -317.1385450321559460 ) ) ;
#74012=CARTESIAN_POINT ( 'NONE',  ( -108.5139559848918367, -295.7099174771433354, -241.8898842515198737 ) ) ;
#74013=CARTESIAN_POINT ( 'NONE',  ( -72.10836744950326249, -292.4070185617318316, -201.8232849165753748 ) ) ;
#74014=CARTESIAN_POINT ( 'NONE',  ( 34.40316898700486803, -293.6905211723409934, -242.4254207124098457 ) ) ;
#74015=CARTESIAN_POINT ( 'NONE',  ( -74.98142758465684210, -291.7027069911534340, -207.7541127260791711 ) ) ;
#74018=CARTESIAN_POINT ( 'NONE',  ( -59.80484286905655011, -299.6247338728821887, -197.9482555088488027 ) ) ;
#74019=CARTESIAN_POINT ( 'NONE',  ( -5.266476787068576471, -273.2598862934049748, -200.7968400251429841 ) ) ;
#74022=CARTESIAN_POINT ( 'NONE',  ( -11.89246028269889521, -276.2373537007119353, -343.0245947462095728 ) ) ;
#74023=CARTESIAN_POINT ( 'NONE',  ( -48.98174036788562802, -272.3014056643684739, -197.4331210636979677 ) ) ;
#74024=CARTESIAN_POINT ( 'NONE',  ( -110.7092802395923030, -280.2657719315449185, -281.6776399509125213 ) ) ;
#74025=CARTESIAN_POINT ( 'NONE',  ( 10.44132800435818176, -274.5237536264277765, -327.1735083567404558 ) ) ;
#74026=CARTESIAN_POINT ( 'NONE',  ( -102.8938401618347598, -298.2042568843719437, -237.2320412923612309 ) ) ;
#74027=CARTESIAN_POINT ( 'NONE',  ( -109.8173900607150273, -273.6363086341236226, -259.4935747174474727 ) ) ;
#74028=CARTESIAN_POINT ( 'NONE',  ( 29.88879290598534411, -300.4807074052612279, -194.1431463050642492 ) ) ;
#74029=CARTESIAN_POINT ( 'NONE',  ( -70.65253295767170982, -271.6351552179695545, -202.7682542806483923 ) ) ;
#74030=CARTESIAN_POINT ( 'NONE',  ( -18.18581442662500791, -295.4500627239226560, -340.9085822236979766 ) ) ;
#74031=CARTESIAN_POINT ( 'NONE',  ( 13.32186135899736712, -291.3526097137193460, -216.9890423849845433 ) ) ;
#74033=CARTESIAN_POINT ( 'NONE',  ( -65.06703844468856346, -277.8970583573882891, -342.1866575937361858 ) ) ;
#74034=CARTESIAN_POINT ( 'NONE',  ( 20.68023803851075115, -275.0956008965272872, -226.0409415048833921 ) ) ;
#74035=CARTESIAN_POINT ( 'NONE',  ( -107.7797056379767042, -282.8528943729294269, -300.3594966493653828 ) ) ;
#74036=CARTESIAN_POINT ( 'NONE',  ( -80.79070720895846591, -297.6399208026963379, -331.7615506574988444 ) ) ;
#74038=CARTESIAN_POINT ( 'NONE',  ( -68.83520217444021227, -284.8243469092976738, -204.3112403664440251 ) ) ;
#74039=CARTESIAN_POINT ( 'NONE',  ( -107.5986887696888914, -282.2038508086868092, -297.2267664648894083 ) ) ;
#74040=CARTESIAN_POINT ( 'NONE',  ( -111.2935362167384028, -276.7527542278039618, -273.3777303605774591 ) ) ;
#74041=CARTESIAN_POINT ( 'NONE',  ( -109.3450387087716678, -276.9280324707634691, -285.5563195962548093 ) ) ;
#74042=CARTESIAN_POINT ( 'NONE',  ( 6.497960560500725791, -282.6475964659681495, -209.4448455354399812 ) ) ;
#74043=CARTESIAN_POINT ( 'NONE',  ( -27.25069010524445901, -275.3881972586881943, -197.6098607496846000 ) ) ;
#74045=CARTESIAN_POINT ( 'NONE',  ( -68.49812611553188901, -272.0494656572178087, -200.8075507593206055 ) ) ;
#74046=CARTESIAN_POINT ( 'NONE',  ( -78.91844335957073042, -281.4937130275479831, -207.6775619331630480 ) ) ;
#74048=CARTESIAN_POINT ( 'NONE',  ( -7.926708649766956327, -288.3545367623178777, -200.7061602810057366 ) ) ;
#74050=CARTESIAN_POINT ( 'NONE',  ( -70.12307423234990722, -287.4837946938689583, -337.8316282302185414 ) ) ;
#74051=CARTESIAN_POINT ( 'NONE',  ( 82.12347693879148380, -301.5478687382300222, -195.3203844934047311 ) ) ;
#74052=CARTESIAN_POINT ( 'NONE',  ( -34.44493754159675802, -296.8841301922085449, -196.9646518883128010 ) ) ;
#74053=CARTESIAN_POINT ( 'NONE',  ( -109.8746062731175925, -288.4859813781841353, -286.2267237104661035 ) ) ;
#74054=CARTESIAN_POINT ( 'NONE',  ( 197.2116108777964030, 281.1590520725322335, -110.1526527170710921 ) ) ;
#74055=CARTESIAN_POINT ( 'NONE',  ( -34.35568795768310935, -296.0893742577463286, -195.3621272966507263 ) ) ;
#74056=CARTESIAN_POINT ( 'NONE',  ( 38.65517597159660568, -286.1187184660389562, -277.2300752977436673 ) ) ;
#74057=CARTESIAN_POINT ( 'NONE',  ( -73.11585798146181503, -283.8248703265669519, -203.2641755041348404 ) ) ;
#74058=CARTESIAN_POINT ( 'NONE',  ( -107.3952957145899489, -290.8242974950010193, -249.7864196659722609 ) ) ;
#74059=CARTESIAN_POINT ( 'NONE',  ( 9.638876423637331214, -282.1382749288294463, -213.6537281136629929 ) ) ;
#74060=CARTESIAN_POINT ( 'NONE',  ( 33.60967859368582822, -282.1193723256164958, -252.4635796065689419 ) ) ;
#74061=CARTESIAN_POINT ( 'NONE',  ( -110.3226172204161060, -292.2914602069034800, -289.1794629474961198 ) ) ;
#74062=AXIS2_PLACEMENT_3D ( 'NONE', #63052, #56403, #57345 ) ;
#74063=CARTESIAN_POINT ( 'NONE',  ( 19.38657721681793333, -298.9107079942916698, -193.3595438923215113 ) ) ;
#74065=CARTESIAN_POINT ( 'NONE',  ( -77.39423046762806280, -287.6643403369684506, -334.4932875205238929 ) ) ;
#74066=CARTESIAN_POINT ( 'NONE',  ( 38.49210793758086879, -275.3842445764277045, -256.9353631442095320 ) ) ;
#74068=CARTESIAN_POINT ( 'NONE',  ( 16.03440785392185930, -294.7929590593000171, -218.1062932318696710 ) ) ;
#74070=CARTESIAN_POINT ( 'NONE',  ( 35.77081079830085031, -283.8376638359844719, -253.6410175316879361 ) ) ;
#74071=CARTESIAN_POINT ( 'NONE',  ( -56.48237439469045285, -275.2979696095242161, -343.1036746451746353 ) ) ;
#74073=CARTESIAN_POINT ( 'NONE',  ( -77.76067872853617757, -295.9187959603378317, -205.7643178802415491 ) ) ;
#74074=CARTESIAN_POINT ( 'NONE',  ( -31.32306011502545573, -273.4787235356348560, -197.4947024048278763 ) ) ;
#74075=CARTESIAN_POINT ( 'NONE',  ( -102.2446926663671434, -291.5994798883600083, -305.3735453317185602 ) ) ;
#74076=CARTESIAN_POINT ( 'NONE',  ( -70.33742643559412500, -292.5473594625576652, -204.9800007217740472 ) ) ;
#74077=CARTESIAN_POINT ( 'NONE',  ( -92.28835985056018387, -287.0133692145570876, -220.6991060442264541 ) ) ;
#74078=CARTESIAN_POINT ( 'NONE',  ( -6.144246839916199576, -293.8793714446516105, -200.5950576397290774 ) ) ;
#74079=CARTESIAN_POINT ( 'NONE',  ( 17.12666970094143082, -294.1239784272474935, -216.5604260796218341 ) ) ;
#74080=CARTESIAN_POINT ( 'NONE',  ( 33.44554181360330603, -293.6208820830340755, -288.1983370152443058 ) ) ;
#74081=CARTESIAN_POINT ( 'NONE',  ( 34.17317958005470757, -289.2602468526873167, -247.7212091064836272 ) ) ;
#74082=CARTESIAN_POINT ( 'NONE',  ( 37.54886640620244265, -281.9433491754959391, -288.3171717360264665 ) ) ;
#74083=CARTESIAN_POINT ( 'NONE',  ( -9.741444982281025844, -296.4749431538819522, -194.8100556288417522 ) ) ;
#74084=CARTESIAN_POINT ( 'NONE',  ( -100.9952947267095311, -284.9579023370150708, -226.9400380962346446 ) ) ;
#74085=CARTESIAN_POINT ( 'NONE',  ( 24.39892694632474601, -276.9611834918085265, -228.3865420773499295 ) ) ;
#74087=CARTESIAN_POINT ( 'NONE',  ( -81.70645854460470048, -284.2274422445447044, -211.8897684659552851 ) ) ;
#74088=CARTESIAN_POINT ( 'NONE',  ( 37.36499653700855106, -285.4597184632267499, -263.1749040344540163 ) ) ;
#74089=CARTESIAN_POINT ( 'NONE',  ( -112.8112183209951951, -276.7839227141478773, -263.1082201134603338 ) ) ;
#74090=CARTESIAN_POINT ( 'NONE',  ( -112.8394912670188432, -266.8193566212495966, -283.2716462811306428 ) ) ;
#74091=CARTESIAN_POINT ( 'NONE',  ( -98.15481678675584476, -284.6214697438447843, -229.8672507439929404 ) ) ;
#74092=CARTESIAN_POINT ( 'NONE',  ( 34.22205117453609802, -283.1049434256077575, -297.6857994496793367 ) ) ;
#74093=CARTESIAN_POINT ( 'NONE',  ( 38.85548804555890712, -286.7331400490336364, -280.1052448063181259 ) ) ;
#74094=CARTESIAN_POINT ( 'NONE',  ( -6.320047787611907886, -296.3990595258504186, -337.5595636656794341 ) ) ;
#74095=CARTESIAN_POINT ( 'NONE',  ( -105.6194086025502941, -279.7115288435012985, -304.3116333470424024 ) ) ;
#74096=CARTESIAN_POINT ( 'NONE',  ( -25.82755104337161001, -278.2235887362064659, -345.9965768796326984 ) ) ;
#74097=CARTESIAN_POINT ( 'NONE',  ( -109.9042652887385714, -278.2743104563852512, -278.7877087598748744 ) ) ;
#74098=CARTESIAN_POINT ( 'NONE',  ( -87.34373792482682575, -299.3530998771738041, -214.6850491549435276 ) ) ;
#74099=CARTESIAN_POINT ( 'NONE',  ( 14.42574231205511559, -284.7815316515611244, -216.2510939733350597 ) ) ;
#74100=CARTESIAN_POINT ( 'NONE',  ( -112.5670063441248487, -291.9987437865419793, -282.5099335869472270 ) ) ;
#74101=CARTESIAN_POINT ( 'NONE',  ( -61.12640126555984210, -294.2885130424811564, -339.7583732013938516 ) ) ;
#74103=CARTESIAN_POINT ( 'NONE',  ( 34.34432392533349798, -293.4021767407929815, -284.2608101467076267 ) ) ;
#74104=CARTESIAN_POINT ( 'NONE',  ( -112.6241767957439208, -291.8163863148431005, -255.6624973926950872 ) ) ;
#74105=CARTESIAN_POINT ( 'NONE',  ( -96.49305964120316048, -279.8038530137138196, -227.4075461153082642 ) ) ;
#74106=CARTESIAN_POINT ( 'NONE',  ( -113.6275033766746816, -271.7183020747088449, -261.7997842456563262 ) ) ;
#74107=CARTESIAN_POINT ( 'NONE',  ( 9.741791337865567613, -287.3326975390622238, -209.5626178559400046 ) ) ;
#74109=CARTESIAN_POINT ( 'NONE',  ( 10.21821628200788723, -288.7500546430942450, -330.9582543885248924 ) ) ;
#74110=CARTESIAN_POINT ( 'NONE',  ( -94.97636106151357183, -285.5172047747840338, -225.5040721867185880 ) ) ;
#74112=CARTESIAN_POINT ( 'NONE',  ( 197.8085509907933499, 288.8371460693426229, -97.00402988771099899 ) ) ;
#74113=CARTESIAN_POINT ( 'NONE',  ( -107.9091210890304922, -264.1399593486416393, -305.3610597610020818 ) ) ;
#74114=CARTESIAN_POINT ( 'NONE',  ( -51.32173023620880059, -276.4326623318781344, -342.1744905856324408 ) ) ;
#74115=CARTESIAN_POINT ( 'NONE',  ( -56.69495985702592833, -276.2277734727795178, -341.1222383648528762 ) ) ;
#74116=CARTESIAN_POINT ( 'NONE',  ( -113.5227515574856199, -272.3617025945729893, -258.9436525938332920 ) ) ;
#74117=CARTESIAN_POINT ( 'NONE',  ( 7.421282116121920680, -59.95783495620983672, -352.0918686609887231 ) ) ;
#74118=CARTESIAN_POINT ( 'NONE',  ( -109.2788355681009591, -276.9041559917061477, -296.5612820402409966 ) ) ;
#74119=CARTESIAN_POINT ( 'NONE',  ( -30.65746628350342107, -296.7288736711072943, -346.0532247793873353 ) ) ;
#74120=CARTESIAN_POINT ( 'NONE',  ( 4.533786936460485251, -293.1263665521543658, -210.4289775808706793 ) ) ;
#74121=CARTESIAN_POINT ( 'NONE',  ( -100.6234947798112529, -297.9318373175615307, -226.7538968511926214 ) ) ;
#74122=CARTESIAN_POINT ( 'NONE',  ( -90.09896791709276442, -273.9815612777582601, -214.3421386863742271 ) ) ;
#74123=CARTESIAN_POINT ( 'NONE',  ( -105.9864616521684439, -296.3861943176669342, -295.3471470798364180 ) ) ;
#74126=CARTESIAN_POINT ( 'NONE',  ( -40.96428677039318700, -281.9270822897667585, -194.8750545159856813 ) ) ;
#74129=CARTESIAN_POINT ( 'NONE',  ( -24.54999144379014098, -282.4008824602091181, -346.2828319175758338 ) ) ;
#74130=CARTESIAN_POINT ( 'NONE',  ( -103.4036249863241039, -279.2022535986235425, -302.2597875590351464 ) ) ;
#74131=CARTESIAN_POINT ( 'NONE',  ( -71.10024695211329515, -279.2517252425743095, -338.4370647884793470 ) ) ;
#74132=CIRCLE ( 'NONE', #80156, 6.654241149514406040 ) ;
#74133=CARTESIAN_POINT ( 'NONE',  ( -54.35297439646813444, -272.3095128412138592, -198.6580894672950421 ) ) ;
#74136=CARTESIAN_POINT ( 'NONE',  ( -43.75320516041123398, -280.1356946007289821, -197.5929865935247278 ) ) ;
#74137=CARTESIAN_POINT ( 'NONE',  ( 25.93972252484041974, -276.9326244026899531, -314.0378611791103367 ) ) ;
#74138=CARTESIAN_POINT ( 'NONE',  ( 9.302661250104792501, -278.4119172560397146, -329.1582303168679573 ) ) ;
#74139=CARTESIAN_POINT ( 'NONE',  ( 23.88455896225976005, -274.7397553729381912, -316.0771052533010561 ) ) ;
#74142=CARTESIAN_POINT ( 'NONE',  ( 37.64409719623136397, -283.6337449956719752, -278.3192184821394903 ) ) ;
#74143=CARTESIAN_POINT ( 'NONE',  ( -77.33489659352031254, -290.6976595528046801, -209.0981931161518617 ) ) ;
#74145=CARTESIAN_POINT ( 'NONE',  ( 38.87534378137304003, -286.7728627327135200, -260.1496046652058567 ) ) ;
#74146=CARTESIAN_POINT ( 'NONE',  ( -109.0808821390584313, -282.5550031631399293, -288.5672647534580051 ) ) ;
#74147=CARTESIAN_POINT ( 'NONE',  ( 14.32556134786536539, -280.8835305204922861, -322.8338868396316457 ) ) ;
#74148=CARTESIAN_POINT ( 'NONE',  ( 27.63605345376637956, -285.1435730492021321, -233.9347213795768994 ) ) ;
#74149=CARTESIAN_POINT ( 'NONE',  ( -35.66905315835412438, -281.2786454423715554, -196.9706347262064696 ) ) ;
#74150=CARTESIAN_POINT ( 'NONE',  ( -110.4869523937869644, -270.7648327691349550, -253.7848480562450106 ) ) ;
#74151=CARTESIAN_POINT ( 'NONE',  ( -49.98108835201040279, -281.6105708526275748, -345.5588711938694360 ) ) ;
#74152=CARTESIAN_POINT ( 'NONE',  ( -11.71597919749275007, -296.7187942265700258, -340.9025581638647964 ) ) ;
#74153=CARTESIAN_POINT ( 'NONE',  ( -103.2192761891207340, -278.7740643137713619, -302.1647717303428067 ) ) ;
#74154=CARTESIAN_POINT ( 'NONE',  ( -102.4651287664665915, -287.0533518826933914, -232.7213364136994755 ) ) ;
#74156=CARTESIAN_POINT ( 'NONE',  ( -94.58627324178790730, -293.1511046174771309, -221.0222393547170441 ) ) ;
#74157=CARTESIAN_POINT ( 'NONE',  ( -13.16411792140720571, -274.7380510624283829, -341.4117965440746048 ) ) ;
#74158=CARTESIAN_POINT ( 'NONE',  ( -34.68266843584159176, -288.2167057135251866, -347.1536200344426106 ) ) ;
#74159=CARTESIAN_POINT ( 'NONE',  ( 34.21682604564620789, -292.1876656275298956, -288.4115403876330106 ) ) ;
#74161=CARTESIAN_POINT ( 'NONE',  ( -106.7353611553109687, -276.9153732991545098, -294.7181068949386145 ) ) ;
#74162=CARTESIAN_POINT ( 'NONE',  ( -102.5636530326079736, -294.2158886811116076, -305.8147826327883081 ) ) ;
#74163=CARTESIAN_POINT ( 'NONE',  ( -92.77272076091672659, -291.1831901360292818, -318.6931876558040244 ) ) ;
#74166=CARTESIAN_POINT ( 'NONE',  ( 10.69745547976779321, -291.1818454733262342, -211.0061316691098625 ) ) ;
#74167=CARTESIAN_POINT ( 'NONE',  ( 24.18992803154551297, -288.5919580142817154, -229.5218649911083730 ) ) ;
#74168=CARTESIAN_POINT ( 'NONE',  ( -83.63106771943982665, -289.6671792578274562, -210.0348093011902222 ) ) ;
#74169=CARTESIAN_POINT ( 'NONE',  ( 32.83002768453177822, -288.6854514182113576, -248.1535970871363190 ) ) ;
#74171=CARTESIAN_POINT ( 'NONE',  ( 29.57688611577420801, -288.7535752083965122, -300.0588731016520114 ) ) ;
#74172=CARTESIAN_POINT ( 'NONE',  ( 21.89469560021595385, -296.1686814398810270, -316.9592505720563054 ) ) ;
#74174=CARTESIAN_POINT ( 'NONE',  ( -9.692263026995922459, -289.9039067114023851, -341.8000243749643801 ) ) ;
#74175=CARTESIAN_POINT ( 'NONE',  ( -28.39472212691228847, -278.1850952643001733, -195.4864586905876820 ) ) ;
#74176=CARTESIAN_POINT ( 'NONE',  ( -114.2106668508827170, -278.8339957343091555, -274.4728385972733236 ) ) ;
#74177=CARTESIAN_POINT ( 'NONE',  ( -33.91196636635813633, -279.7609149242800868, -193.4587043800007962 ) ) ;
#74178=CARTESIAN_POINT ( 'NONE',  ( -105.2246696219695679, -298.9429321745295738, -239.1923035306274983 ) ) ;
#74179=CARTESIAN_POINT ( 'NONE',  ( -111.3918456094949505, -282.7058103652747718, -258.3813427142728187 ) ) ;
#74181=CARTESIAN_POINT ( 'NONE',  ( 10.08355039165451394, -278.8531153773471942, -213.1826983043261237 ) ) ;
#74182=CARTESIAN_POINT ( 'NONE',  ( -80.43381689840293802, -281.6355078497830959, -331.8089213787535527 ) ) ;
#74184=CARTESIAN_POINT ( 'NONE',  ( 25.48492106058643714, -274.6100447701479652, -313.7598548026060143 ) ) ;
#74185=CARTESIAN_POINT ( 'NONE',  ( -71.23258788700917421, -297.0281155915316731, -335.8131086055824426 ) ) ;
#74186=CARTESIAN_POINT ( 'NONE',  ( -27.42574595424867212, -281.8494419526655292, -346.4613967982887743 ) ) ;
#74187=CARTESIAN_POINT ( 'NONE',  ( -102.9737209920723870, -297.0529721176575890, -302.9694683793557033 ) ) ;
#74188=CARTESIAN_POINT ( 'NONE',  ( -29.14231603631001732, -299.4679527596301227, -193.8524759526805497 ) ) ;
#74189=CARTESIAN_POINT ( 'NONE',  ( -1.708603960716748027, -274.2049357877133957, -206.6100763448369548 ) ) ;
#74190=CARTESIAN_POINT ( 'NONE',  ( -2.735465052274779207, -294.5098884657392091, -203.8223387212208024 ) ) ;
#74191=CARTESIAN_POINT ( 'NONE',  ( 37.50491720582801491, -287.9456423537644696, -288.4995206869028834 ) ) ;
#74192=CARTESIAN_POINT ( 'NONE',  ( -11.96942020510595484, -278.4595397325391559, -199.1334162389412654 ) ) ;
#74193=CARTESIAN_POINT ( 'NONE',  ( -104.6089459959524817, -290.8712549167677253, -232.8895602642143388 ) ) ;
#74195=CARTESIAN_POINT ( 'NONE',  ( -10.64947778649820798, -287.7541318172500837, -338.6132590646933522 ) ) ;
#74196=CARTESIAN_POINT ( 'NONE',  ( 5.378483930638676469, -290.6302035946492310, -208.7170872873702479 ) ) ;
#74199=CARTESIAN_POINT ( 'NONE',  ( -98.89698570470234529, -289.5158858671409803, -309.7176328080411167 ) ) ;
#74202=CARTESIAN_POINT ( 'NONE',  ( -33.75036370400606955, -287.0375576705206413, -193.6804651681037797 ) ) ;
#74203=CARTESIAN_POINT ( 'NONE',  ( 7.399455738971494334, -289.1948066931273615, -214.2051214447836571 ) ) ;
#74204=CARTESIAN_POINT ( 'NONE',  ( -61.52883221686803239, -294.4174750897554986, -343.2713593892869994 ) ) ;
#74205=CARTESIAN_POINT ( 'NONE',  ( 15.42559372803626694, -283.6399427132246274, -325.7588703823795981 ) ) ;
#74206=CARTESIAN_POINT ( 'NONE',  ( -108.4257852916168474, -284.1656393340111890, -287.0305788076659610 ) ) ;
#74207=CARTESIAN_POINT ( 'NONE',  ( 34.60067056430946053, -276.6697423702598257, -255.2817985388676334 ) ) ;
#74208=CARTESIAN_POINT ( 'NONE',  ( 17.97365442908223443, -290.8692873434143848, -220.1648392913227497 ) ) ;
#74209=CARTESIAN_POINT ( 'NONE',  ( -3.910196677923111430, -273.2982361392400890, -205.0058636741025566 ) ) ;
#74211=CARTESIAN_POINT ( 'NONE',  ( 82.64890176555634582, -299.5541904835127980, -193.4639945212225882 ) ) ;
#74212=CARTESIAN_POINT ( 'NONE',  ( -57.81342177691675488, -287.7060124194463242, -198.7377550460897453 ) ) ;
#74213=CARTESIAN_POINT ( 'NONE',  ( -102.8444006202213501, -297.1088799957351512, -310.2470645987006037 ) ) ;
#74214=CARTESIAN_POINT ( 'NONE',  ( -96.66239236556258163, -285.8003595659675966, -227.6203485177996697 ) ) ;
#74215=CARTESIAN_POINT ( 'NONE',  ( -86.95229483053950048, -276.7816050235325633, -329.0106157297087179 ) ) ;
#74216=CARTESIAN_POINT ( 'NONE',  ( -3.373863047587286168, -293.1402728206653023, -201.3574793792092237 ) ) ;
#74217=CARTESIAN_POINT ( 'NONE',  ( 30.56957947083360949, -286.1318155425817054, -304.0704878820728823 ) ) ;
#74218=CARTESIAN_POINT ( 'NONE',  ( -13.78447876091214930, -295.0878441723444894, -343.6468711199851782 ) ) ;
#74219=CARTESIAN_POINT ( 'NONE',  ( -95.13372741009565914, -291.5136508546605683, -225.7273967675308768 ) ) ;
#74222=CARTESIAN_POINT ( 'NONE',  ( 202.9738562182569694, 291.9636489450776367, -53.99999999998589573 ) ) ;
#74223=CARTESIAN_POINT ( 'NONE',  ( -110.2692008201007212, -286.3588767831299720, -247.7267792911372339 ) ) ;
#74224=CARTESIAN_POINT ( 'NONE',  ( 99.50465036329318025, -297.2649936051624309, -195.4191791630918829 ) ) ;
#74226=CARTESIAN_POINT ( 'NONE',  ( -16.05582445442620099, -281.6906413642141160, -340.5119381469079372 ) ) ;
#74227=CARTESIAN_POINT ( 'NONE',  ( -109.7183351150041943, -277.8858906361336949, -296.7347603891257677 ) ) ;
#74228=CARTESIAN_POINT ( 'NONE',  ( 37.17548521243185178, -283.4568815351546505, -262.9449483833741397 ) ) ;
#74229=CARTESIAN_POINT ( 'NONE',  ( -53.95492635066413101, -170.5480224260624595, -362.9304601937118946 ) ) ;
#74230=CARTESIAN_POINT ( 'NONE',  ( -47.19846773905869952, -281.7497809990708788, -346.1334772183409996 ) ) ;
#74231=CARTESIAN_POINT ( 'NONE',  ( -37.25418869707253577, -284.0733264649528564, -195.7036466603310316 ) ) ;
#74232=CARTESIAN_POINT ( 'NONE',  ( -41.15469939162760227, -275.8651894647484255, -194.6409025646760540 ) ) ;
#74233=CARTESIAN_POINT ( 'NONE',  ( -109.7980990638689889, -297.1732283303375084, -260.5947241346065084 ) ) ;
#74234=CARTESIAN_POINT ( 'NONE',  ( 4.080622000029026530, -293.1657283542152754, -331.0688992511239803 ) ) ;
#74235=CARTESIAN_POINT ( 'NONE',  ( -110.5670492534069638, -278.9059964574320247, -294.0135811907408083 ) ) ;
#74236=CARTESIAN_POINT ( 'NONE',  ( 23.98438602724380075, -276.1014720859656109, -310.0537069353559900 ) ) ;
#74237=CARTESIAN_POINT ( 'NONE',  ( -99.32537813508778868, -274.2346074061051127, -225.1120375430513150 ) ) ;
#74238=CARTESIAN_POINT ( 'NONE',  ( -96.82340113892685451, -276.8200872927554883, -318.7905676282600211 ) ) ;
#74239=CARTESIAN_POINT ( 'NONE',  ( 199.3883137936200001, 289.5528945227777058, -97.47147507494776164 ) ) ;
#74240=CARTESIAN_POINT ( 'NONE',  ( -88.15956483509424402, -275.7628482977409021, -325.5901777202634548 ) ) ;
#74241=CARTESIAN_POINT ( 'NONE',  ( -27.80325290580884001, -296.3586970821630757, -346.2270913909829346 ) ) ;
#74244=CARTESIAN_POINT ( 'NONE',  ( -109.8017535281590114, -285.4814158217897671, -281.8114575661990102 ) ) ;
#74245=CARTESIAN_POINT ( 'NONE',  ( -113.3275550324223957, -286.3167537601562458, -270.0091723368642533 ) ) ;
#74246=CARTESIAN_POINT ( 'NONE',  ( 28.90582449703376966, -286.4840023110999141, -239.4554850190929756 ) ) ;
#74247=CARTESIAN_POINT ( 'NONE',  ( -97.04098497541068014, -277.5526752548092304, -226.9740714690790071 ) ) ;
#74248=CARTESIAN_POINT ( 'NONE',  ( -107.7106542079722686, -286.7233110525971256, -246.5552194900701863 ) ) ;
#74249=CARTESIAN_POINT ( 'NONE',  ( -34.26518688321827000, -278.5713711660569629, -196.7193659866738074 ) ) ;
#74250=CARTESIAN_POINT ( 'NONE',  ( -26.96422480088653373, -277.9967704120463168, -342.9320080064891840 ) ) ;
#74252=CARTESIAN_POINT ( 'NONE',  ( -71.94240322811519661, -274.0743634838763114, -205.9558532541948068 ) ) ;
#74253=CARTESIAN_POINT ( 'NONE',  ( 38.71289882921283976, -282.4921885438012623, -281.3090309299198566 ) ) ;
#74254=CARTESIAN_POINT ( 'NONE',  ( 26.22622989088633005, -281.4713161893278084, -226.9248280585386226 ) ) ;
#74255=ORIENTED_EDGE ( 'NONE', *, *, #17187, .F. ) ;
#74258=CARTESIAN_POINT ( 'NONE',  ( 2.077802800986792153, -288.4343977221430464, -205.6586584570499099 ) ) ;
#74259=CARTESIAN_POINT ( 'NONE',  ( -72.91647737234427495, -296.7650176620357456, -206.4311801504561004 ) ) ;
#74261=CARTESIAN_POINT ( 'NONE',  ( -50.54069270061050645, -291.2364138903745356, -194.6042741902552393 ) ) ;
#74262=CARTESIAN_POINT ( 'NONE',  ( 20.89355311358891854, -286.6623060109966445, -315.5408491286260073 ) ) ;
#74263=CARTESIAN_POINT ( 'NONE',  ( 31.94815039128375744, -286.4542466626979262, -295.1460232981478953 ) ) ;
#74264=CARTESIAN_POINT ( 'NONE',  ( -95.27990595236231286, -286.3888582228834707, -225.2819121754416187 ) ) ;
#74265=CARTESIAN_POINT ( 'NONE',  ( -71.94129019521366786, -275.5093619187966851, -336.9176766755859376 ) ) ;
#74266=CARTESIAN_POINT ( 'NONE',  ( -9.870945756821738470, -287.0991552338770703, -341.4371200483362827 ) ) ;
#74267=CARTESIAN_POINT ( 'NONE',  ( -24.16303721481126843, -288.2204700402649564, -196.4752339651858790 ) ) ;
#74268=CARTESIAN_POINT ( 'NONE',  ( -67.34603664332830419, -287.4445661234304339, -339.2796802088391246 ) ) ;
#74269=CARTESIAN_POINT ( 'NONE',  ( 17.78986660362062011, -283.1789916838747558, -318.5681589442484096 ) ) ;
#74270=CARTESIAN_POINT ( 'NONE',  ( -80.88947172212748171, -293.4626542202238397, -209.0943242593519926 ) ) ;
#74273=CARTESIAN_POINT ( 'NONE',  ( -90.63748525421374325, -299.2240114166103240, -216.7992520273537593 ) ) ;
#74274=CARTESIAN_POINT ( 'NONE',  ( 22.25094745951394160, -280.1577587267901777, -227.9191802236357489 ) ) ;
#74275=CARTESIAN_POINT ( 'NONE',  ( 19.09344709063815060, -280.2380545062007400, -319.7582313521128299 ) ) ;
#74276=CARTESIAN_POINT ( 'NONE',  ( -2.050764562359526089, -293.7940121440358325, -338.6158517957313165 ) ) ;
#74277=CARTESIAN_POINT ( 'NONE',  ( -68.36544722251517214, -296.0375658166813650, -203.3848713452751156 ) ) ;
#74278=CARTESIAN_POINT ( 'NONE',  ( 28.01965655893107865, -274.1101830806572934, -306.0947473372763170 ) ) ;
#74279=CARTESIAN_POINT ( 'NONE',  ( -39.68811552978801416, -296.3973767741737788, -343.8293186784129034 ) ) ;
#74281=CARTESIAN_POINT ( 'NONE',  ( -34.76887997977183886, -296.5636955617469539, -194.0550975974727237 ) ) ;
#74282=CARTESIAN_POINT ( 'NONE',  ( -110.6208171951045216, -294.5368397234319673, -290.4644763386635873 ) ) ;
#74284=CARTESIAN_POINT ( 'NONE',  ( 8.943109179223133864, -293.5086301619486449, -213.6357451189632286 ) ) ;
#74286=CARTESIAN_POINT ( 'NONE',  ( -112.6811021722686235, -282.6131832261027625, -267.1586120766681915 ) ) ;
#74287=CARTESIAN_POINT ( 'NONE',  ( 12.35487423371159821, -294.3371112082193122, -323.9023603761793879 ) ) ;
#74288=CARTESIAN_POINT ( 'NONE',  ( -10.70203441136842493, -282.7142641241646857, -342.6626824732124987 ) ) ;
#74289=CARTESIAN_POINT ( 'NONE',  ( -3.065630858972029138, -282.4214935763112635, -203.0082293663973019 ) ) ;
#74290=CARTESIAN_POINT ( 'NONE',  ( -105.4114129437495535, -284.6844284073017661, -234.2990003802526928 ) ) ;
#74291=CARTESIAN_POINT ( 'NONE',  ( -111.5138416205268754, -288.6846530816837344, -260.0519279142316122 ) ) ;
#74292=CARTESIAN_POINT ( 'NONE',  ( -20.25526795762938548, -274.3380690714490129, -345.3683826091709648 ) ) ;
#74293=CARTESIAN_POINT ( 'NONE',  ( -16.35131107719725208, -281.2656609137384862, -343.7787756204624543 ) ) ;
#74294=CARTESIAN_POINT ( 'NONE',  ( -71.39193019565041709, -284.2773771114291321, -205.2318211071049916 ) ) ;
#74295=CARTESIAN_POINT ( 'NONE',  ( -112.0131427866932796, -289.6920281034611548, -252.8777498112525564 ) ) ;
#74296=CARTESIAN_POINT ( 'NONE',  ( 121.3395553409046670, -299.5541904835127980, -192.6222259952039622 ) ) ;
#74297=CARTESIAN_POINT ( 'NONE',  ( -72.48781540059938777, -297.1256234784556796, -335.2692314726747327 ) ) ;
#74298=CARTESIAN_POINT ( 'NONE',  ( -101.4071785498490641, -280.5296171531674645, -228.6213660314736558 ) ) ;
#74299=CARTESIAN_POINT ( 'NONE',  ( -9.029914148653487516, -292.7039837757203600, -340.2508277693513037 ) ) ;
#74300=CARTESIAN_POINT ( 'NONE',  ( 18.85509418752544164, -280.5576104057058728, -223.7154537223013904 ) ) ;
#74301=CARTESIAN_POINT ( 'NONE',  ( 30.90332604778165049, -294.1788930963834900, -306.0208488668643554 ) ) ;
#74302=CARTESIAN_POINT ( 'NONE',  ( -109.7354827147009360, -282.3547029023094979, -292.0499055703522231 ) ) ;
#74303=CARTESIAN_POINT ( 'NONE',  ( -42.63881503186441790, -279.1191573715983054, -345.1738256140021122 ) ) ;
#74304=CARTESIAN_POINT ( 'NONE',  ( -50.52529040036783670, -294.2834035789922495, -342.4000060569163679 ) ) ;
#74305=CARTESIAN_POINT ( 'NONE',  ( -110.0384582495561432, -270.7993796880480204, -251.0517014249982708 ) ) ;
#74308=CARTESIAN_POINT ( 'NONE',  ( 35.55196497664078237, -283.7394077024633816, -286.4347110644710028 ) ) ;
#74309=CARTESIAN_POINT ( 'NONE',  ( -68.54931480292256651, -294.9812553376125379, -336.4359937688024047 ) ) ;
#74311=CARTESIAN_POINT ( 'NONE',  ( 35.77081079830085031, -279.2666405000204009, -287.0812184334320705 ) ) ;
#74312=CARTESIAN_POINT ( 'NONE',  ( -93.04804104595032754, -272.4743287490172179, -217.4178005367461708 ) ) ;
#74315=CARTESIAN_POINT ( 'NONE',  ( 38.29547707787573074, -288.7214397035533011, -258.7711607790917583 ) ) ;
#74316=CARTESIAN_POINT ( 'NONE',  ( -89.81484536658261675, -291.1188366280158561, -219.6110536152962709 ) ) ;
#74317=CARTESIAN_POINT ( 'NONE',  ( -74.87543661120152194, -281.0631348903510229, -206.8837973115952309 ) ) ;
#74318=CARTESIAN_POINT ( 'NONE',  ( -21.78504608824203359, -275.8550072343882107, -198.2193760567121785 ) ) ;
#74319=CARTESIAN_POINT ( 'NONE',  ( -67.45524397145867113, -278.4430546652495195, -203.4123589535383303 ) ) ;
#74320=CARTESIAN_POINT ( 'NONE',  ( 13.11145476838443358, -278.3477951844204199, -325.9246729007232943 ) ) ;
#74321=ORIENTED_EDGE ( 'NONE', *, *, #67056, .T. ) ;
#74322=CARTESIAN_POINT ( 'NONE',  ( -76.43089144562425474, -273.3781816181504496, -203.9592119032449773 ) ) ;
#74323=CARTESIAN_POINT ( 'NONE',  ( -63.32584561161473857, -293.6311159737196022, -200.6034059995096754 ) ) ;
#74326=CARTESIAN_POINT ( 'NONE',  ( -22.41359796218076283, -290.3807676340355783, -196.0280721708947453 ) ) ;
#74327=CARTESIAN_POINT ( 'NONE',  ( -39.16460267741054935, -297.6954021136285178, -197.3503183705244908 ) ) ;
#74328=DIRECTION ( 'NONE',  ( 0.000000000000000000, 0.000000000000000000, 1.000000000000000000 ) ) ;
#74330=CARTESIAN_POINT ( 'NONE',  ( -108.8311409013396656, -292.4144971234878199, -243.5277136732773897 ) ) ;
#74331=CARTESIAN_POINT ( 'NONE',  ( -111.2586520408596868, -298.6233781216987495, -305.9938812882205070 ) ) ;
#74332=CARTESIAN_POINT ( 'NONE',  ( -27.62305892795291129, -288.1760595998777035, -196.1615462988393972 ) ) ;
#74333=CARTESIAN_POINT ( 'NONE',  ( 36.51239812411534302, -273.7112893900501263, -282.7400878787908027 ) ) ;
#74334=CARTESIAN_POINT ( 'NONE',  ( 8.192834175133336672, -276.6007277210825350, -211.4720665324349511 ) ) ;
#74336=CARTESIAN_POINT ( 'NONE',  ( -36.15920225219416295, -290.1469025963456829, -195.9177844392693544 ) ) ;
#74337=CARTESIAN_POINT ( 'NONE',  ( -20.06134422237167669, -282.1321961327722079, -196.5393866169997352 ) ) ;
#74339=CARTESIAN_POINT ( 'NONE',  ( -21.37401719523599297, -282.1906402055314516, -341.7499092765669388 ) ) ;
#74340=CARTESIAN_POINT ( 'NONE',  ( -112.9341364414093789, -279.7942230935132102, -257.4275924630767918 ) ) ;
#74341=CARTESIAN_POINT ( 'NONE',  ( -35.92202204239944052, -281.8296820789292383, -346.9639398720143504 ) ) ;
#74342=CARTESIAN_POINT ( 'NONE',  ( -95.96173002589530654, -278.8233761499683396, -319.9446178456882421 ) ) ;
#74344=CARTESIAN_POINT ( 'NONE',  ( -1.773587678670080603, -278.1096710169149446, -337.8712441191687503 ) ) ;
#74345=CARTESIAN_POINT ( 'NONE',  ( -6.998514795304313196, -282.9805209788415823, -207.2794874003663779 ) ) ;
#74348=CARTESIAN_POINT ( 'NONE',  ( -110.5383651108679430, -298.3424059769417340, -286.7088667224956566 ) ) ;
#74349=CARTESIAN_POINT ( 'NONE',  ( -10.59857451505935266, -289.7747291194127115, -338.6726651190762141 ) ) ;
#74350=CARTESIAN_POINT ( 'NONE',  ( -21.32410925686333414, -274.8659531575454480, -343.3202690396299204 ) ) ;
#74351=CARTESIAN_POINT ( 'NONE',  ( -4.747138555727826947, -290.3888921443942763, -339.0162759747175301 ) ) ;
#74352=CARTESIAN_POINT ( 'NONE',  ( -64.10121037084631723, -291.0422306162756172, -202.3194748939237115 ) ) ;
#74353=CARTESIAN_POINT ( 'NONE',  ( -26.15969992683964307, -288.4210817735253727, -346.4826640427768325 ) ) ;
#74355=CARTESIAN_POINT ( 'NONE',  ( -110.2922948431506285, -282.8020485770121013, -281.8542908167387964 ) ) ;
#74356=CARTESIAN_POINT ( 'NONE',  ( -109.6357122242981035, -292.6320679111305481, -253.4402205839576538 ) ) ;
#74357=CARTESIAN_POINT ( 'NONE',  ( -57.56625575297894670, -284.2662901310447978, -199.4442311161974146 ) ) ;
#74358=CARTESIAN_POINT ( 'NONE',  ( 9.578597816045999025, -282.0281943631513855, -213.7286431888898335 ) ) ;
#74359=CARTESIAN_POINT ( 'NONE',  ( 37.79073451879185086, -288.2950721807467289, -254.5514875830503456 ) ) ;
#74360=CARTESIAN_POINT ( 'NONE',  ( -107.8780378778167091, -278.7931810922888758, -289.4035311347136599 ) ) ;
#74361=CARTESIAN_POINT ( 'NONE',  ( -71.97892723770681300, -290.3994350421806416, -202.0218469895243629 ) ) ;
#74362=CARTESIAN_POINT ( 'NONE',  ( 38.62437946567852265, -288.2091809579479218, -258.7274406370387396 ) ) ;
#74363=CARTESIAN_POINT ( 'NONE',  ( 38.72378295961302541, -287.8987456826200173, -258.7162333983712870 ) ) ;
#74364=CARTESIAN_POINT ( 'NONE',  ( -110.3186946369728503, -284.6755760802865325, -273.6402521901212026 ) ) ;
#74367=CARTESIAN_POINT ( 'NONE',  ( 1.053372854503991762, -294.4188834145718943, -204.9855999183268693 ) ) ;
#74368=CARTESIAN_POINT ( 'NONE',  ( 15.12822800443399629, -293.0147362738269976, -326.0406017586187772 ) ) ;
#74369=CARTESIAN_POINT ( 'NONE',  ( 20.19991521567041204, -275.2481289316073685, -315.6844109011823321 ) ) ;
#74370=CARTESIAN_POINT ( 'NONE',  ( -33.33274563387125511, -297.4497003231595613, -193.4634797602432457 ) ) ;
#74371=CARTESIAN_POINT ( 'NONE',  ( 35.98726964839713105, -291.9299183629871663, -262.5474586246740500 ) ) ;
#74372=CARTESIAN_POINT ( 'NONE',  ( -109.1527491887405148, -295.0258693783389390, -252.3887151296896434 ) ) ;
#74373=CARTESIAN_POINT ( 'NONE',  ( -41.63130488942617546, -293.2021424450839504, -197.0393842864601481 ) ) ;
#74374=CARTESIAN_POINT ( 'NONE',  ( 6.257771624124649712, -295.5244042031038134, -329.3592016807214122 ) ) ;
#74375=CARTESIAN_POINT ( 'NONE',  ( -71.26987233637623831, -293.4989171417172429, -337.4350142532647965 ) ) ;
#74376=CARTESIAN_POINT ( 'NONE',  ( -39.87806681634610584, -300.0204473827804463, -195.4008640690309733 ) ) ;
#74377=CARTESIAN_POINT ( 'NONE',  ( 25.14526171442063784, -287.9688531825754012, -232.1670340492557614 ) ) ;
#74378=CARTESIAN_POINT ( 'NONE',  ( -37.10623521012158932, -279.0290699526048002, -345.7287345265697809 ) ) ;
#74379=CARTESIAN_POINT ( 'NONE',  ( -1.666329217425129849, -275.3849138376474457, -338.1495877242780921 ) ) ;
#74380=CARTESIAN_POINT ( 'NONE',  ( -95.00453865079963123, -272.5905489873999272, -219.4856834363111773 ) ) ;
#74381=CARTESIAN_POINT ( 'NONE',  ( 36.86236028920718155, -279.7166023735151157, -276.9015252067166557 ) ) ;
#74382=CARTESIAN_POINT ( 'NONE',  ( -110.6762066588404991, -276.6898771852445407, -291.0611317095278991 ) ) ;
#74383=CARTESIAN_POINT ( 'NONE',  ( -75.93115960312972845, -294.2636857189538091, -332.9672154734957985 ) ) ;
#74385=CARTESIAN_POINT ( 'NONE',  ( -68.33333082419196103, -274.2854179530394845, -204.1400633143957180 ) ) ;
#74388=CARTESIAN_POINT ( 'NONE',  ( -112.4747267976864720, -288.4901308595647720, -276.7876747164512494 ) ) ;
#74389=CARTESIAN_POINT ( 'NONE',  ( -40.77281631427023711, -273.8412531982428959, -197.3920957385186057 ) ) ;
#74390=CARTESIAN_POINT ( 'NONE',  ( -111.9220341017839786, -290.3118881862409353, -289.5652037930871643 ) ) ;
#74391=CARTESIAN_POINT ( 'NONE',  ( -110.0516000095905298, -274.7990515660800384, -251.1012609257627446 ) ) ;
#74392=CARTESIAN_POINT ( 'NONE',  ( -109.7498088093044686, -294.3080251928071220, -289.3087866927871232 ) ) ;
#74393=CARTESIAN_POINT ( 'NONE',  ( -88.22228193851803724, -282.9402523210974323, -328.0110311091816584 ) ) ;
#74396=CARTESIAN_POINT ( 'NONE',  ( -14.76940321423028735, -280.7596475703621763, -341.9375972552663825 ) ) ;
#74398=CARTESIAN_POINT ( 'NONE',  ( -102.0001744625215565, -288.8747207771212402, -305.2023618553584470 ) ) ;
#74399=CARTESIAN_POINT ( 'NONE',  ( -64.52943918650947808, -281.5504621017586828, -339.4385551503341389 ) ) ;
#74402=CARTESIAN_POINT ( 'NONE',  ( 35.90851475125332826, -291.3444308077713458, -254.1955369459573717 ) ) ;
#74403=CARTESIAN_POINT ( 'NONE',  ( 20.38666278060578563, -276.4315573732993130, -224.5354333153332220 ) ) ;
#74404=CARTESIAN_POINT ( 'NONE',  ( -90.15322104215556465, -284.9836560794788056, -325.9221400664249586 ) ) ;
#74405=CARTESIAN_POINT ( 'NONE',  ( -63.04385334104880911, -271.7998665417416078, -199.3068182006708753 ) ) ;
#74406=CARTESIAN_POINT ( 'NONE',  ( -93.25510141768785388, -285.2186397766125765, -223.4282770688946016 ) ) ;
#74407=CARTESIAN_POINT ( 'NONE',  ( -8.491075900962258061, -278.0922386890936195, -338.0727508235528376 ) ) ;
#74408=CARTESIAN_POINT ( 'NONE',  ( 26.91345581806242748, -276.8327314527761587, -305.4509997985492191 ) ) ;
#74409=CARTESIAN_POINT ( 'NONE',  ( -98.15153259721294887, -285.9536657162455526, -314.3473572246385288 ) ) ;
#74412=CARTESIAN_POINT ( 'NONE',  ( -95.58288815029770547, -295.7050537587094254, -320.7294018751268254 ) ) ;
#74413=CARTESIAN_POINT ( 'NONE',  ( 18.09565210015753678, -288.8318479730476724, -220.3565779592980789 ) ) ;
#74415=CARTESIAN_POINT ( 'NONE',  ( -115.3288506153726871, -288.2666405000203440, -252.5284128619063608 ) ) ;
#74416=CARTESIAN_POINT ( 'NONE',  ( -71.08614568659650956, -278.5375199563519004, -201.4930927078843297 ) ) ;
#74418=CARTESIAN_POINT ( 'NONE',  ( 10.63111465465473948, -291.1018519268682212, -211.0897586184356953 ) ) ;
#74419=CARTESIAN_POINT ( 'NONE',  ( -97.93697271887768352, -286.6513227032351097, -228.3993158769825698 ) ) ;
#74420=CARTESIAN_POINT ( 'NONE',  ( -67.74273012630460755, -281.4077920386654341, -202.8658312501284229 ) ) ;
#74421=CARTESIAN_POINT ( 'NONE',  ( -33.77314354132587226, -287.5214997728434128, -194.0337199024757240 ) ) ;
#74422=CARTESIAN_POINT ( 'NONE',  ( -1.449737705333953519, -284.5764642520662164, -336.2299405513745114 ) ) ;
#74423=CARTESIAN_POINT ( 'NONE',  ( 27.64996968141183231, -276.2611344248434762, -311.7528824236853211 ) ) ;
#74424=CARTESIAN_POINT ( 'NONE',  ( -68.71638578619146642, -295.6578635449241119, -202.6162392225266728 ) ) ;
#74425=CARTESIAN_POINT ( 'NONE',  ( -71.23268171405550220, -279.4503635259903263, -201.2206712695470117 ) ) ;
#74426=CARTESIAN_POINT ( 'NONE',  ( -82.84327368075298637, -299.3449638387971845, -211.3812500184892826 ) ) ;
#74428=CARTESIAN_POINT ( 'NONE',  ( 31.95455697924148097, -277.6233781216988064, -236.9535640164627637 ) ) ;
#74429=CARTESIAN_POINT ( 'NONE',  ( -65.06756053210973789, -295.8334655272168447, -199.7956035823811760 ) ) ;
#74431=CARTESIAN_POINT ( 'NONE',  ( -109.3478020360252998, -277.8957349463242963, -282.8088541779085858 ) ) ;
#74432=CARTESIAN_POINT ( 'NONE',  ( -34.13525353535147389, -275.2967092788854870, -193.8253262272209554 ) ) ;
#74433=CARTESIAN_POINT ( 'NONE',  ( 29.55096314886815989, -281.1022398462984597, -308.1283107966947910 ) ) ;
#74434=CARTESIAN_POINT ( 'NONE',  ( 24.36657668382832043, -289.8718390835347805, -311.2506764947798956 ) ) ;
#74435=CARTESIAN_POINT ( 'NONE',  ( -36.21675946851736683, -299.5861093703725828, -194.0541616449634432 ) ) ;
#74436=CARTESIAN_POINT ( 'NONE',  ( -108.0028001540073603, -297.3774787112935201, -300.0790362160719269 ) ) ;
#74437=CARTESIAN_POINT ( 'NONE',  ( -33.43763853027527233, -294.1015478300986388, -195.6168812054621924 ) ) ;
#74438=CARTESIAN_POINT ( 'NONE',  ( 37.25436919034387984, -279.6366088427694763, -276.9369696465074639 ) ) ;
#74439=CARTESIAN_POINT ( 'NONE',  ( -16.54233966998446448, -282.2431711383076163, -198.8859418724097452 ) ) ;
#74440=CARTESIAN_POINT ( 'NONE',  ( -52.91290239512851912, -295.9310171204095923, -197.5149993817916538 ) ) ;
#74441=CARTESIAN_POINT ( 'NONE',  ( -111.7395502861892567, -285.9440777478470181, -286.8353496933402198 ) ) ;
#74442=CARTESIAN_POINT ( 'NONE',  ( -18.40686695056283995, -287.7228650447567588, -341.2355177415550997 ) ) ;
#74443=CARTESIAN_POINT ( 'NONE',  ( -54.80317017044318106, -170.1808862240834799, -364.2540321147021132 ) ) ;
#74445=CARTESIAN_POINT ( 'NONE',  ( -9.792831157893585825, -287.2739831076702899, -341.6328943831270522 ) ) ;
#74446=CARTESIAN_POINT ( 'NONE',  ( -33.23322400512102348, -285.7718862169706995, -197.4058112397049740 ) ) ;
#74448=CARTESIAN_POINT ( 'NONE',  ( -99.52971831975739292, -285.0333253451539122, -315.3290480821412984 ) ) ;
#74449=CARTESIAN_POINT ( 'NONE',  ( 35.72006355777654107, -275.9015243157707005, -271.5810856146622427 ) ) ;
#74450=CARTESIAN_POINT ( 'NONE',  ( -16.69655938608546109, -291.2331300248984576, -196.5013138080821307 ) ) ;
#74451=CARTESIAN_POINT ( 'NONE',  ( 36.88444105832943620, -281.9510129430772736, -250.2166081798807227 ) ) ;
#74452=CARTESIAN_POINT ( 'NONE',  ( 33.67201438717807349, -282.7134019369103726, -242.2928093641701821 ) ) ;
#74453=CARTESIAN_POINT ( 'NONE',  ( -8.043001199000883616, -283.0121296584449055, -341.6028280931179779 ) ) ;
#74454=CARTESIAN_POINT ( 'NONE',  ( -4.347568898116098701, -280.4995962340121878, -205.2289706140603585 ) ) ;
#74455=CARTESIAN_POINT ( 'NONE',  ( -69.85430415644619018, -277.1237833571632905, -202.7746430608542312 ) ) ;
#74456=CARTESIAN_POINT ( 'NONE',  ( -39.19203910876188957, -139.8860650072662395, -364.8865173942490401 ) ) ;
#74459=CARTESIAN_POINT ( 'NONE',  ( 35.28238792420321346, -277.3199673538305206, -252.3120109468044916 ) ) ;
#74460=CARTESIAN_POINT ( 'NONE',  ( 120.7794652203165384, 149.8366910277294721, -263.1582692822088916 ) ) ;
#74461=VECTOR ( 'NONE', #93174, 1000.000000000000000 ) ;
#74462=CARTESIAN_POINT ( 'NONE',  ( -102.6196269175759568, -296.3480666490015096, -237.3442557441241263 ) ) ;
#74463=CARTESIAN_POINT ( 'NONE',  ( 19.37454105035772400, -292.3519631758443325, -218.3727068714760264 ) ) ;
#74464=CARTESIAN_POINT ( 'NONE',  ( 6.721591756639591075, -59.76906970966732757, -351.2517004600837254 ) ) ;
#74467=CARTESIAN_POINT ( 'NONE',  ( -113.3707211231467795, -271.3444403225931296, -261.8237742107333474 ) ) ;
#74468=CARTESIAN_POINT ( 'NONE',  ( -111.1068926226098625, -288.9054794258566972, -273.9275184348696257 ) ) ;
#74469=CARTESIAN_POINT ( 'NONE',  ( -41.07808676104863821, -296.9600592232346798, -344.5150127863178113 ) ) ;
#74470=CARTESIAN_POINT ( 'NONE',  ( -54.89021727451788735, -287.1371130972721062, -198.9411534029229358 ) ) ;
#74472=CARTESIAN_POINT ( 'NONE',  ( 25.52885602376467489, -295.0778638287242757, -314.4307816401636728 ) ) ;
#74474=CARTESIAN_POINT ( 'NONE',  ( -70.23702101035104306, -283.9901133535744293, -335.6122621973509013 ) ) ;
#74475=CARTESIAN_POINT ( 'NONE',  ( -30.51309233569872958, -296.9307883448980192, -193.7595496953030931 ) ) ;
#74476=CARTESIAN_POINT ( 'NONE',  ( -88.54949493537256444, -292.1580181088114614, -213.0730688708309515 ) ) ;
#74477=CARTESIAN_POINT ( 'NONE',  ( 24.84024731074108772, -294.6465772469834974, -315.6926085923652749 ) ) ;
#74478=CARTESIAN_POINT ( 'NONE',  ( -101.6421408529779455, -290.2462557845285005, -305.0291504973097858 ) ) ;
#74481=CARTESIAN_POINT ( 'NONE',  ( -77.56705765604836245, -299.3787824471317549, -206.1565535717396358 ) ) ;
#74482=CARTESIAN_POINT ( 'NONE',  ( -60.73518434341271188, -272.5502855448310129, -197.3622829227206807 ) ) ;
#74483=CARTESIAN_POINT ( 'NONE',  ( 31.57194632179529492, -280.9417072537235640, -295.2964247345689728 ) ) ;
#74485=CARTESIAN_POINT ( 'NONE',  ( -7.913978800448858486, -276.1844590866720068, -341.4636183676226437 ) ) ;
#74486=CARTESIAN_POINT ( 'NONE',  ( -36.70896333572505199, -272.4601010954729645, -196.5512761557083650 ) ) ;
#74487=CARTESIAN_POINT ( 'NONE',  ( -110.4993787953527118, -280.2481180415809945, -283.0384786833326984 ) ) ;
#74488=CARTESIAN_POINT ( 'NONE',  ( -16.04886409159475136, -274.9135922770327056, -341.5309844200425573 ) ) ;
#74489=CARTESIAN_POINT ( 'NONE',  ( -73.05342960719087841, -298.7726017082547969, -206.2377768113724130 ) ) ;
#74490=CARTESIAN_POINT ( 'NONE',  ( -93.10069673837531923, -274.1667385059606659, -222.8618366217195330 ) ) ;
#74491=CARTESIAN_POINT ( 'NONE',  ( -70.97471974561103991, -275.3745832571113965, -202.2230668747978655 ) ) ;
#74492=CARTESIAN_POINT ( 'NONE',  ( 21.49037822252698149, -272.9275879052044047, -223.2535638062848307 ) ) ;
#74493=CARTESIAN_POINT ( 'NONE',  ( 20.25809048107894839, -293.5697321689932551, -225.3280041404554481 ) ) ;
#74494=CARTESIAN_POINT ( 'NONE',  ( 7.045982686199225853, -291.2449697668599811, -211.6660710887996117 ) ) ;
#74496=CARTESIAN_POINT ( 'NONE',  ( -80.18670820232593144, -278.1074201805467396, -334.3301169551698990 ) ) ;
#74497=CARTESIAN_POINT ( 'NONE',  ( -29.99197734301977292, -274.3144461314024625, -197.7320495630668518 ) ) ;
#74498=CARTESIAN_POINT ( 'NONE',  ( -94.97434894510037395, -282.5521186816318391, -320.6778752702667816 ) ) ;
#74500=CARTESIAN_POINT ( 'NONE',  ( 35.33075626097016908, -295.7985704219074705, -289.5637873726855673 ) ) ;
#74502=EDGE_CURVE ( 'NONE', #72158, #16725, #42301, .T. ) ;
#74503=CARTESIAN_POINT ( 'NONE',  ( -93.37219179858823281, -284.4159370588170077, -223.3166100077042415 ) ) ;
#74504=CARTESIAN_POINT ( 'NONE',  ( -112.3799589767046143, -282.4853212626185268, -275.5648646428933830 ) ) ;
#74505=CARTESIAN_POINT ( 'NONE',  ( 29.62976360303615664, -273.7175100886929613, -239.7386353479813863 ) ) ;
#74506=CARTESIAN_POINT ( 'NONE',  ( 0.6748366296861562086, -282.5591208869451521, -205.6953921195959083 ) ) ;
#74507=CARTESIAN_POINT ( 'NONE',  ( 30.65163309939041980, -277.1270872422682601, -298.1376447020237492 ) ) ;
#74510=CARTESIAN_POINT ( 'NONE',  ( -73.54660511883022878, -271.9802241836293319, -203.2528950018933642 ) ) ;
#74511=CARTESIAN_POINT ( 'NONE',  ( -48.20328226370995850, -279.1900778561374068, -344.7915089576744094 ) ) ;
#74513=CARTESIAN_POINT ( 'NONE',  ( -43.57237465170776858, -287.8943063226583376, -195.0061790519320084 ) ) ;
#74514=CARTESIAN_POINT ( 'NONE',  ( -46.33728359802502439, -287.1659958044081122, -344.8709239999969327 ) ) ;
#74516=CARTESIAN_POINT ( 'NONE',  ( -100.2291351389269352, -295.8661852229679425, -232.4165611199517514 ) ) ;
#74517=CARTESIAN_POINT ( 'NONE',  ( -45.52169314129997701, -287.2964876897261206, -344.1442677779785413 ) ) ;
#74518=CARTESIAN_POINT ( 'NONE',  ( 196.7899183121812712, 289.3460118731243824, -81.74456998406768093 ) ) ;
#74520=CARTESIAN_POINT ( 'NONE',  ( 29.74383084652408371, -286.5079753812884178, -306.8341827236661175 ) ) ;
#74521=CARTESIAN_POINT ( 'NONE',  ( -10.66781026394506959, -284.2986247113133800, -339.2262223411310629 ) ) ;
#74522=CARTESIAN_POINT ( 'NONE',  ( -37.33711657186668731, -281.2919249635348820, -346.3606807609200473 ) ) ;
#74523=CARTESIAN_POINT ( 'NONE',  ( -107.0016159787469689, -290.8419565030084186, -248.4902171929243764 ) ) ;
#74525=CARTESIAN_POINT ( 'NONE',  ( -5.318355093415077839, -281.9073318073209862, -204.1049462552673219 ) ) ;
#74526=CARTESIAN_POINT ( 'NONE',  ( -4.746056831878517457, -283.4142233113976204, -335.8601696216384767 ) ) ;
#74528=CARTESIAN_POINT ( 'NONE',  ( -86.29633191721167407, -291.7070242071380335, -327.7170751631025496 ) ) ;
#74530=CARTESIAN_POINT ( 'NONE',  ( -65.54398275188748357, -297.8602344018348731, -198.6547647197295987 ) ) ;
#74533=CARTESIAN_POINT ( 'NONE',  ( 34.99953025153173769, -285.9115961641270474, -292.2248193765338442 ) ) ;
#74534=CARTESIAN_POINT ( 'NONE',  ( 30.54306557180798265, -276.0231117972085144, -306.8145663582024554 ) ) ;
#74535=CARTESIAN_POINT ( 'NONE',  ( -5.359256051990131553, -294.4549278816123206, -202.9009752452699615 ) ) ;
#74537=CARTESIAN_POINT ( 'NONE',  ( -4.829096099716510437, -288.9805209788416391, -202.7746430608542312 ) ) ;
#74539=CARTESIAN_POINT ( 'NONE',  ( -38.54185504977358079, -275.0670126259199151, -345.5182071940267292 ) ) ;
#74541=CARTESIAN_POINT ( 'NONE',  ( -62.56086652396250258, -296.1292289337201282, -198.4553876069790022 ) ) ;
#74542=CARTESIAN_POINT ( 'NONE',  ( -109.2111646212260894, -292.3718225183703225, -253.5363135654050666 ) ) ;
#74543=CARTESIAN_POINT ( 'NONE',  ( -24.57048249866506495, -273.5678994651693756, -198.3317608097948437 ) ) ;
#74545=CARTESIAN_POINT ( 'NONE',  ( -110.1005841813927617, -291.9183737462051340, -282.1387600919331362 ) ) ;
#74546=CARTESIAN_POINT ( 'NONE',  ( -90.93953621487675321, -292.2088467961463607, -220.4358557993474790 ) ) ;
#74547=CARTESIAN_POINT ( 'NONE',  ( -96.72150534157410107, -285.7010192338174761, -314.5427063229685700 ) ) ;
#74548=CARTESIAN_POINT ( 'NONE',  ( -37.80977384094381932, -293.4716626462308113, -193.9517782229605416 ) ) ;
#74549=CARTESIAN_POINT ( 'NONE',  ( -83.97907833090116014, -292.7419996236841939, -209.6457327047583021 ) ) ;
#74550=CARTESIAN_POINT ( 'NONE',  ( 31.53934685475475419, -293.7089098982257838, -294.6868567051899959 ) ) ;
#74551=CARTESIAN_POINT ( 'NONE',  ( 25.19072945925428542, -290.1118196254051895, -311.7934739645593254 ) ) ;
#74552=CARTESIAN_POINT ( 'NONE',  ( 2.095961023225290543, -282.7060421323228070, -336.4948528492595301 ) ) ;
#74553=CARTESIAN_POINT ( 'NONE',  ( -36.18671901538648683, -296.1463551561196823, -194.8014844089030646 ) ) ;
#74554=CARTESIAN_POINT ( 'NONE',  ( -110.9253999516530200, -284.6723469387944760, -247.5004223799076328 ) ) ;
#74556=CARTESIAN_POINT ( 'NONE',  ( 36.74167249923987555, -277.6552678733329458, -279.9123376469342475 ) ) ;
#74558=CARTESIAN_POINT ( 'NONE',  ( -109.3153428794948070, -283.5358074838680977, -255.9762212167196935 ) ) ;
#74559=CARTESIAN_POINT ( 'NONE',  ( 34.77536254014806616, -285.2848066338809758, -249.5820697348338797 ) ) ;
#74560=CARTESIAN_POINT ( 'NONE',  ( -86.31512814432410607, -275.8625889891196721, -328.2390265326181407 ) ) ;
#74561=CARTESIAN_POINT ( 'NONE',  ( -36.19885267344637469, -282.5450916471686469, -343.4137178100369852 ) ) ;
#74563=CARTESIAN_POINT ( 'NONE',  ( -86.56139755788984758, -280.5912267190093417, -211.5941817532333573 ) ) ;
#74564=CARTESIAN_POINT ( 'NONE',  ( 20.38801330599852690, -287.2977451278451326, -320.9783517006832767 ) ) ;
#74565=CARTESIAN_POINT ( 'NONE',  ( -0.2307040938277708231, -296.3118910867993350, -334.4567036891482985 ) ) ;
#74566=CARTESIAN_POINT ( 'NONE',  ( -3.066506567493172408, -278.2071212142495824, -338.4318830179549309 ) ) ;
#74567=CARTESIAN_POINT ( 'NONE',  ( 23.13856152000264998, -277.4971963590528503, -317.2378529591339316 ) ) ;
#74568=CARTESIAN_POINT ( 'NONE',  ( -92.72802326105372117, -277.7084412444256145, -317.9148267163085961 ) ) ;
#74569=CARTESIAN_POINT ( 'NONE',  ( -98.39281327570978419, -299.1417535791921978, -227.0853740671206253 ) ) ;
#74570=CARTESIAN_POINT ( 'NONE',  ( 36.37782344695926895, -285.3826938240433151, -257.2051224602344064 ) ) ;
#74571=CARTESIAN_POINT ( 'NONE',  ( -41.69428031497560738, -290.7062168319934585, -346.4497932967893234 ) ) ;
#74573=CARTESIAN_POINT ( 'NONE',  ( -55.89476207235227179, -294.2168998337880907, -341.3362892187378748 ) ) ;
#74575=CARTESIAN_POINT ( 'NONE',  ( 24.44288267907244006, -293.7574771579027129, -309.3759162100105300 ) ) ;
#74576=ORIENTED_EDGE ( 'NONE', *, *, #23269, .F. ) ;
#74577=CARTESIAN_POINT ( 'NONE',  ( -38.90005457043210413, -290.1509399999799257, -347.0361728722741645 ) ) ;
#74578=CARTESIAN_POINT ( 'NONE',  ( -68.57435866483670850, -280.2819038159683487, -204.2671416360386445 ) ) ;
#74579=CARTESIAN_POINT ( 'NONE',  ( -54.51253556097567099, -296.7568374629867094, -195.6171890023048263 ) ) ;
#74580=CARTESIAN_POINT ( 'NONE',  ( 22.33130144436584175, -288.8553181748212637, -318.8838615061009136 ) ) ;
#74582=CARTESIAN_POINT ( 'NONE',  ( -40.33368669971463305, -289.4220480538710945, -347.2948845676187375 ) ) ;
#74583=CARTESIAN_POINT ( 'NONE',  ( -67.78931714311427470, -283.7964223850520398, -336.7315188022645884 ) ) ;
#74584=CARTESIAN_POINT ( 'NONE',  ( -78.20562432208285486, -208.4051219816803098, -357.1155072845333507 ) ) ;
#74585=CARTESIAN_POINT ( 'NONE',  ( 63.31788037795879376, 48.12403318353134551, -317.4058823860502230 ) ) ;
#74586=CARTESIAN_POINT ( 'NONE',  ( 192.4389841540552766, 276.2114567146547301, -124.0227208457718575 ) ) ;
#74587=CARTESIAN_POINT ( 'NONE',  ( -93.73702429105561862, -277.0898851584242948, -316.9872856407504287 ) ) ;
#74588=CARTESIAN_POINT ( 'NONE',  ( -110.7013089757634958, -277.4690012365063012, -270.6255046054959053 ) ) ;
#74589=CARTESIAN_POINT ( 'NONE',  ( -35.46747341460690706, -297.5826843317813655, -193.4228076759506223 ) ) ;
#74590=CARTESIAN_POINT ( 'NONE',  ( -29.16725854433003917, -125.6520135956795343, -361.6366667242135122 ) ) ;
#74591=CARTESIAN_POINT ( 'NONE',  ( -70.10512885389582038, -276.1595777985966151, -339.5119668820257175 ) ) ;
#74593=CARTESIAN_POINT ( 'NONE',  ( -108.7214969898345203, -290.8383632685606131, -286.0049216929098179 ) ) ;
#74594=CARTESIAN_POINT ( 'NONE',  ( -37.61736449087290168, -298.8516106606287508, -193.5230881369411406 ) ) ;
#74595=CARTESIAN_POINT ( 'NONE',  ( 35.00421311571506067, -286.4064624732968696, -283.2960441815861827 ) ) ;
#74596=CARTESIAN_POINT ( 'NONE',  ( 7.937813434781497257, -299.0971729166703881, -193.4189769336720985 ) ) ;
#74597=CARTESIAN_POINT ( 'NONE',  ( -110.3743096031691806, -296.7402843377415138, -268.7350142468995386 ) ) ;
#74601=CARTESIAN_POINT ( 'NONE',  ( -61.91414478594938231, -279.2891147995922552, -341.8692121690097565 ) ) ;
#74602=CARTESIAN_POINT ( 'NONE',  ( 31.01959451852300731, -281.5152315338775679, -305.6635300432021722 ) ) ;
#74605=CARTESIAN_POINT ( 'NONE',  ( -107.9196266286643890, -279.8933075908891510, -250.4907771230259641 ) ) ;
#74606=CARTESIAN_POINT ( 'NONE',  ( -106.5061940358336017, -280.7213068450871560, -238.7661636572613304 ) ) ;
#74607=CARTESIAN_POINT ( 'NONE',  ( -37.80818305410353020, -296.6209222390689888, -196.7733655183099586 ) ) ;
#74609=CARTESIAN_POINT ( 'NONE',  ( -76.82364142031509857, -279.6742897887572781, -208.8990965991897042 ) ) ;
#74611=CARTESIAN_POINT ( 'NONE',  ( -101.0803355052465946, -273.9225869453792939, -227.3531469752605005 ) ) ;
#74612=CARTESIAN_POINT ( 'NONE',  ( -30.05910102807533590, -276.1444902714620753, -195.7155260257193277 ) ) ;
#74613=CARTESIAN_POINT ( 'NONE',  ( 37.64403716789804832, -273.9417716245968109, -255.6728404604151592 ) ) ;
#74617=CARTESIAN_POINT ( 'NONE',  ( -69.07841855503879458, -290.8209576393734892, -204.4277702186211627 ) ) ;
#74618=CARTESIAN_POINT ( 'NONE',  ( -109.8783495895170574, -284.2232261030928839, -244.8317766016182020 ) ) ;
#74619=CARTESIAN_POINT ( 'NONE',  ( 22.61990526554245307, -280.3909596132652382, -313.7715161841854865 ) ) ;
#74620=CARTESIAN_POINT ( 'NONE',  ( 34.33842590173269826, -279.9089483340678157, -253.7077564161002101 ) ) ;
#74621=CARTESIAN_POINT ( 'NONE',  ( -82.32979142192327515, -283.5124790073619465, -211.0535650343738610 ) ) ;
#74622=CARTESIAN_POINT ( 'NONE',  ( 14.64436009215091516, -290.3209326453991821, -324.4914692580782685 ) ) ;
#74623=CARTESIAN_POINT ( 'NONE',  ( 33.49277846266131320, -282.5040700248410417, -251.0879014629102244 ) ) ;
#74625=CARTESIAN_POINT ( 'NONE',  ( -66.29138683552255884, -281.8247395054848994, -340.8617248607095007 ) ) ;
#74626=CARTESIAN_POINT ( 'NONE',  ( 37.60914795013002987, -295.5871765860491678, -273.0760798960645843 ) ) ;
#74628=CARTESIAN_POINT ( 'NONE',  ( -28.32273446397356764, -278.4048108225163105, -194.8586629213227752 ) ) ;
#74629=CARTESIAN_POINT ( 'NONE',  ( -24.13369580814710957, -288.2204700384499461, -196.3110530287767119 ) ) ;
#74631=CARTESIAN_POINT ( 'NONE',  ( -87.70815786347243659, -293.2751597080068677, -214.0358649360418610 ) ) ;
#74633=CARTESIAN_POINT ( 'NONE',  ( 36.08447192361377631, -273.3549442812906705, -255.0144107655211201 ) ) ;
#74634=CARTESIAN_POINT ( 'NONE',  ( -17.77533050566854911, -288.0031866045580387, -344.6666763198309695 ) ) ;
#74635=CARTESIAN_POINT ( 'NONE',  ( 35.99959510425156139, -292.0650627557170083, -279.0244636905586049 ) ) ;
#74637=CARTESIAN_POINT ( 'NONE',  ( 7.870682762519501274, -275.1048211780591259, -328.3663010028109284 ) ) ;
#74638=CARTESIAN_POINT ( 'NONE',  ( -109.3677199865572049, -294.9256108842549793, -252.3336631719506045 ) ) ;
#74639=CARTESIAN_POINT ( 'NONE',  ( -61.40074955970969484, -290.6864848932543168, -339.8046606485491452 ) ) ;
#74641=FACE_OUTER_BOUND ( 'NONE', #7962, .T. ) ;
#74642=CARTESIAN_POINT ( 'NONE',  ( 31.56824404916997651, -291.6067402642401589, -237.4643740468311819 ) ) ;
#74643=CARTESIAN_POINT ( 'NONE',  ( -11.76361223995900929, -287.9909596785881831, -201.1353869647859938 ) ) ;
#74644=CARTESIAN_POINT ( 'NONE',  ( -82.27175383587551494, -287.8958367020495643, -331.6413291870662192 ) ) ;
#74645=CARTESIAN_POINT ( 'NONE',  ( 29.33625009638695857, -288.5603536269874212, -239.2255134550925106 ) ) ;
#74647=CARTESIAN_POINT ( 'NONE',  ( 26.50331050835565350, -287.8661213482336620, -234.5305204014277649 ) ) ;
#74649=CARTESIAN_POINT ( 'NONE',  ( -14.26133472441101446, -296.7341899374411582, -342.0946773094296418 ) ) ;
#74651=CARTESIAN_POINT ( 'NONE',  ( -21.08328019671219167, -287.4613720088320861, -195.5034363540314075 ) ) ;
#74652=CARTESIAN_POINT ( 'NONE',  ( -92.30367283701568226, -275.9098965787842417, -322.2869320629129106 ) ) ;
#74653=CARTESIAN_POINT ( 'NONE',  ( -69.00279887320714067, -277.7904995120650256, -340.5418856368893898 ) ) ;
#74655=CARTESIAN_POINT ( 'NONE',  ( -41.00314227784342336, -279.6740111104205653, -193.4561961316451573 ) ) ;
#74656=CARTESIAN_POINT ( 'NONE',  ( -111.7826102751215842, -274.5079294519437667, -267.6079199030569953 ) ) ;
#74657=CARTESIAN_POINT ( 'NONE',  ( -74.52566161415958845, -283.5574047903530186, -205.2128744216350924 ) ) ;
#74659=CARTESIAN_POINT ( 'NONE',  ( -19.21031484309129311, -278.4273714888736890, -198.3210066536638294 ) ) ;
#74660=CARTESIAN_POINT ( 'NONE',  ( -34.57883112759889599, -281.0172621181535533, -345.3102154168523725 ) ) ;
#74662=CARTESIAN_POINT ( 'NONE',  ( 28.48795114482039992, -274.5389194072199643, -308.9508156319882914 ) ) ;
#74663=CARTESIAN_POINT ( 'NONE',  ( -110.0437901406154850, -297.9148625708127156, -282.4074394538689035 ) ) ;
#74664=CARTESIAN_POINT ( 'NONE',  ( -69.07116951183981257, -282.3800769487669413, -340.1947658067326188 ) ) ;
#74665=CARTESIAN_POINT ( 'NONE',  ( -93.80262519537068044, -298.1526680131651688, -223.6985741638340244 ) ) ;
#74666=CARTESIAN_POINT ( 'NONE',  ( -57.27746367952408235, -299.1154359049074856, -196.4423722683945641 ) ) ;
#74667=CARTESIAN_POINT ( 'NONE',  ( -69.49644856640914270, -273.2835449454844365, -204.8007668567211113 ) ) ;
#74668=CARTESIAN_POINT ( 'NONE',  ( 24.59875578216602676, -296.1260809153042715, -312.7412272011486607 ) ) ;
#74669=CARTESIAN_POINT ( 'NONE',  ( 28.69745350106223114, -287.2012906447548630, -230.6624547502133566 ) ) ;
#74670=CARTESIAN_POINT ( 'NONE',  ( -108.2462714497051337, -276.9700567163104097, -244.0978233810913025 ) ) ;
#74671=CARTESIAN_POINT ( 'NONE',  ( -110.4302280783941228, -290.6923369096060696, -245.9648077804576474 ) ) ;
#74673=CARTESIAN_POINT ( 'NONE',  ( -106.2580277091146570, -289.2819623090607593, -295.1390969273053315 ) ) ;
#74674=CARTESIAN_POINT ( 'NONE',  ( 37.24519107588339750, -291.6590403477949280, -278.6985173699114853 ) ) ;
#74675=ORIENTED_EDGE ( 'NONE', *, *, #90226, .F. ) ;
#74676=CARTESIAN_POINT ( 'NONE',  ( -78.59295187722810283, -208.2960365483323244, -357.4574221067172743 ) ) ;
#74677=CARTESIAN_POINT ( 'NONE',  ( 20.40224211447447544, -287.6899141941705693, -315.1432481485496737 ) ) ;
#74679=CARTESIAN_POINT ( 'NONE',  ( -111.6441841938612356, -285.2506829658910874, -289.6994918278102205 ) ) ;
#74680=CARTESIAN_POINT ( 'NONE',  ( 8.719349482866910250, -291.7246806358665481, -208.8846716486493165 ) ) ;
#74681=CARTESIAN_POINT ( 'NONE',  ( 38.18373531343226546, -283.0221040040140679, -282.6580890615919657 ) ) ;
#74682=CARTESIAN_POINT ( 'NONE',  ( 9.907080499280741748, -282.2135394191683986, -326.0742696650880816 ) ) ;
#74683=CARTESIAN_POINT ( 'NONE',  ( -57.38971816702794371, -297.8004735578203963, -195.9615257826633297 ) ) ;
#74685=CARTESIAN_POINT ( 'NONE',  ( 21.06330951981307464, -276.2439090687676071, -225.7298909334321593 ) ) ;
#74686=CARTESIAN_POINT ( 'NONE',  ( -44.43188863514384224, -289.9822598732267807, -196.0018478709972669 ) ) ;
#74687=CARTESIAN_POINT ( 'NONE',  ( -19.15849291125192977, -273.0861830429902284, -199.1993213799163698 ) ) ;
#74690=CARTESIAN_POINT ( 'NONE',  ( -60.44838011321432703, -287.6703021060756100, -199.5981648483642061 ) ) ;
#74691=AXIS2_PLACEMENT_3D ( 'NONE', #1857, #61037, #16531 ) ;
#74692=CARTESIAN_POINT ( 'NONE',  ( -113.4696086260547503, -297.7482906846398691, -261.0856634291062051 ) ) ;
#74694=CARTESIAN_POINT ( 'NONE',  ( -107.4550924571893944, -285.4790225035231401, -249.4972071373100846 ) ) ;
#74695=CARTESIAN_POINT ( 'NONE',  ( -113.5342344903518921, -277.4882595307880138, -280.1376066241720082 ) ) ;
#74696=CARTESIAN_POINT ( 'NONE',  ( 37.36296280046943963, -294.4325920663882812, -288.6515394447459357 ) ) ;
#74697=CARTESIAN_POINT ( 'NONE',  ( 29.06060803431240913, -285.2103190098962955, -233.7687920394562298 ) ) ;
#74698=CARTESIAN_POINT ( 'NONE',  ( -1.973414832039259714, -294.9299421931800680, -338.7338368609741792 ) ) ;
#74699=CARTESIAN_POINT ( 'NONE',  ( -74.72308090585572415, -289.8978238285169482, -333.1031539349582431 ) ) ;
#74700=CARTESIAN_POINT ( 'NONE',  ( 144.7857639756989272, -299.5541904835127980, -195.3611179825600175 ) ) ;
#74701=CIRCLE ( 'NONE', #71754, 3.491568894204821749 ) ;
#74703=CARTESIAN_POINT ( 'NONE',  ( 65.27003054854583297, 46.14720179368438835, -315.3780817363856954 ) ) ;
#74704=CARTESIAN_POINT ( 'NONE',  ( -82.87778781722306576, -286.9624316419063916, -209.0647282615439337 ) ) ;
#74705=CARTESIAN_POINT ( 'NONE',  ( -69.85430415644619018, -295.1237833571632905, -202.7746430608542312 ) ) ;
#74707=CARTESIAN_POINT ( 'NONE',  ( -107.2848808473092248, -283.1826639939407073, -292.3196594784668605 ) ) ;
#74708=CARTESIAN_POINT ( 'NONE',  ( -109.5848754348886587, -278.5566739754412424, -243.6240218369687511 ) ) ;
#74709=CARTESIAN_POINT ( 'NONE',  ( 34.73187271808695442, -283.8119169376137734, -290.4963737698603268 ) ) ;
#74710=CARTESIAN_POINT ( 'NONE',  ( 47.10975143806707877, 10.86743066051956674, -330.5726880037435649 ) ) ;
#74711=CARTESIAN_POINT ( 'NONE',  ( -95.83108803412343946, -282.4595386525951426, -319.5504424561300993 ) ) ;
#74712=CARTESIAN_POINT ( 'NONE',  ( 10.09475186357033571, -284.7299907931557073, -212.7275355671475836 ) ) ;
#74713=CARTESIAN_POINT ( 'NONE',  ( -82.85727382234014726, -275.2979259275561503, -209.7261570950452665 ) ) ;
#74715=CARTESIAN_POINT ( 'NONE',  ( -23.50103805800856449, -295.3629202040891641, -342.1513509979731111 ) ) ;
#74716=CARTESIAN_POINT ( 'NONE',  ( 9.173829443841141185, -291.3909643450470526, -213.3956335164136817 ) ) ;
#74717=CARTESIAN_POINT ( 'NONE',  ( -99.56239595340080939, -278.6029753664799387, -315.5708686191259176 ) ) ;
#74718=CARTESIAN_POINT ( 'NONE',  ( 32.09818047943307562, -275.8509181170630882, -292.8800651429879167 ) ) ;
#74719=CARTESIAN_POINT ( 'NONE',  ( 39.39793777515723860, -274.4827912382892237, -271.1821122752888868 ) ) ;
#74721=CARTESIAN_POINT ( 'NONE',  ( 22.14339226843788921, -274.1785583418645160, -316.1226970260628946 ) ) ;
#74722=CARTESIAN_POINT ( 'NONE',  ( -32.03517119519862177, -296.4117396034024523, -346.6005595134861892 ) ) ;
#74725=CARTESIAN_POINT ( 'NONE',  ( -90.95819938144680350, -284.9158675454273180, -320.3560885456327583 ) ) ;
#74726=CARTESIAN_POINT ( 'NONE',  ( -34.49420280291450069, -284.7769559991329515, -346.2944161767139235 ) ) ;
#74727=CARTESIAN_POINT ( 'NONE',  ( -27.81506604715598030, -285.5249131026939722, -197.8825976396125270 ) ) ;
#74728=CARTESIAN_POINT ( 'NONE',  ( -79.10128632590647157, -276.0253444707420840, -331.2721642435360536 ) ) ;
#74729=CARTESIAN_POINT ( 'NONE',  ( 35.15167481083326351, -283.6199507831899496, -286.3478647997922053 ) ) ;
#74730=CARTESIAN_POINT ( 'NONE',  ( -103.7642556815463735, -276.6028785229590312, -302.3971499174763835 ) ) ;
#74731=CARTESIAN_POINT ( 'NONE',  ( -68.15488413106277221, -278.5462484948705537, -336.8938952929489687 ) ) ;
#74733=CARTESIAN_POINT ( 'NONE',  ( -8.930341675178043559, -281.2173108727161548, -198.9681664298150281 ) ) ;
#74734=CARTESIAN_POINT ( 'NONE',  ( -7.566598880602133370, -280.9244873450692239, -199.4033969406857238 ) ) ;
#74738=CARTESIAN_POINT ( 'NONE',  ( 37.07247553566636356, -289.2315434154735954, -256.1190695676899622 ) ) ;
#74740=CARTESIAN_POINT ( 'NONE',  ( -106.8570136222426754, -296.0532736473377327, -247.3921832803019356 ) ) ;
#74741=CARTESIAN_POINT ( 'NONE',  ( -96.49513449550056521, -290.5625199193334538, -221.2064256652056997 ) ) ;
#74742=CARTESIAN_POINT ( 'NONE',  ( 36.32215744010836289, -286.0771094970806985, -273.8114135028199030 ) ) ;
#74743=CARTESIAN_POINT ( 'NONE',  ( 16.42919824622496705, -286.8444008847733357, -320.6757354959104873 ) ) ;
#74744=CARTESIAN_POINT ( 'NONE',  ( -83.91159045529833804, -286.6012890637580313, -213.5643399303619674 ) ) ;
#74745=CARTESIAN_POINT ( 'NONE',  ( -59.10951669156793997, -275.3337007887078585, -342.1327196678263363 ) ) ;
#74746=CARTESIAN_POINT ( 'NONE',  ( 14.04898559246379364, -286.7452795909547945, -326.6948265027494358 ) ) ;
#74748=CARTESIAN_POINT ( 'NONE',  ( 25.44904982844451169, -288.9990628942607032, -229.3449947107535536 ) ) ;
#74749=CARTESIAN_POINT ( 'NONE',  ( -15.50967131853788672, -286.7702195614238576, -342.3418241194708571 ) ) ;
#74750=CARTESIAN_POINT ( 'NONE',  ( 34.46374763106584282, -282.6835988905652925, -284.8251852979579439 ) ) ;
#74751=CARTESIAN_POINT ( 'NONE',  ( -110.4729343686655625, -292.3290191794417865, -287.7899739523396647 ) ) ;
#74752=CARTESIAN_POINT ( 'NONE',  ( 82.12354321084184505, -301.5426637435585349, -195.0595354636311924 ) ) ;
#74755=CARTESIAN_POINT ( 'NONE',  ( -111.4806179995697732, -298.6590389822279690, -255.7090317016075289 ) ) ;
#74756=CARTESIAN_POINT ( 'NONE',  ( -19.48526938302004297, -279.4847846655044350, -199.3597877154836624 ) ) ;
#74757=CARTESIAN_POINT ( 'NONE',  ( 20.00765610291796648, -280.2205166870371045, -318.7137670881525651 ) ) ;
#74758=CARTESIAN_POINT ( 'NONE',  ( 39.34024589018421381, -292.8204604414252117, -276.0374227009869514 ) ) ;
#74759=CARTESIAN_POINT ( 'NONE',  ( -35.77407587660231769, -296.4719660400812700, -196.5615479667378054 ) ) ;
#74760=CARTESIAN_POINT ( 'NONE',  ( 34.97984321487042791, -273.8607736341372174, -288.0473391452588885 ) ) ;
#74761=CARTESIAN_POINT ( 'NONE',  ( -35.62239879105807461, -296.3453436971453243, -343.8467374541819481 ) ) ;
#74763=CARTESIAN_POINT ( 'NONE',  ( 30.04588848858884731, -297.3612107378443739, -194.0714852076413592 ) ) ;
#74765=CARTESIAN_POINT ( 'NONE',  ( -112.6514675479462824, -294.6588674810529938, -280.8672498933675001 ) ) ;
#74767=CARTESIAN_POINT ( 'NONE',  ( -44.37444271633743398, -293.3868752960044048, -197.0574800988244704 ) ) ;
#74769=CARTESIAN_POINT ( 'NONE',  ( 35.45491819872999884, -294.2524986060451511, -262.5745906210389649 ) ) ;
#74771=CARTESIAN_POINT ( 'NONE',  ( -109.3467057471019217, -282.8594273508513197, -247.9666385871875320 ) ) ;
#74772=CARTESIAN_POINT ( 'NONE',  ( -53.14937721894284550, -295.2603851840459583, -341.6810290768895015 ) ) ;
#74774=CARTESIAN_POINT ( 'NONE',  ( -63.91201610298173819, -283.3892812254445630, -342.6315705132724929 ) ) ;
#74775=CARTESIAN_POINT ( 'NONE',  ( 5.350128041316613903, -282.5451605733809970, -208.0175376922692863 ) ) ;
#74776=CARTESIAN_POINT ( 'NONE',  ( -67.17694600861631216, -285.3382476379308628, -199.3991394672190154 ) ) ;
#74777=CARTESIAN_POINT ( 'NONE',  ( -111.7944044328310724, -288.6489923936499054, -262.8229984059123581 ) ) ;
#74778=CARTESIAN_POINT ( 'NONE',  ( 1.722420631277537195, -281.0195122186840422, -335.9103530788731291 ) ) ;
#74779=TOROIDAL_SURFACE ( 'NONE', #29372, 5.343514653206205445, 0.5000000000000000000 ) ;
#74780=CARTESIAN_POINT ( 'NONE',  ( -44.05284660852944967, -284.6503451611625906, -197.1750264699281558 ) ) ;
#74781=CARTESIAN_POINT ( 'NONE',  ( 38.48204486032361871, -286.3269807973474599, -258.7734843738759309 ) ) ;
#74783=CARTESIAN_POINT ( 'NONE',  ( 23.60505849873323214, -295.7261133713067807, -312.0670162002215307 ) ) ;
#74784=CARTESIAN_POINT ( 'NONE',  ( -111.8314114925341869, -280.1919948465773587, -253.3349852269796827 ) ) ;
#74785=CARTESIAN_POINT ( 'NONE',  ( -66.31583001594192694, -293.4496828956232548, -339.9372684927440105 ) ) ;
#74786=CARTESIAN_POINT ( 'NONE',  ( -100.8280979475137116, -278.7128352065659556, -234.2839121786687713 ) ) ;
#74787=CARTESIAN_POINT ( 'NONE',  ( 39.60696130180528485, -293.7539912578243388, -273.1724359357992853 ) ) ;
#74788=CIRCLE ( 'NONE', #33717, 5.343514653206204557 ) ;
#74789=CARTESIAN_POINT ( 'NONE',  ( -106.5963192455231621, -283.0260877451271426, -240.0126481903064359 ) ) ;
#74790=CARTESIAN_POINT ( 'NONE',  ( -64.35042687199577927, -279.4046283875090353, -340.3839925747799953 ) ) ;
#74791=CARTESIAN_POINT ( 'NONE',  ( -9.151351836338086798, -293.7330361916733068, -337.9670199209332395 ) ) ;
#74792=CARTESIAN_POINT ( 'NONE',  ( -48.64280816747923808, -295.9082238641929052, -196.1651650767377646 ) ) ;
#74795=CARTESIAN_POINT ( 'NONE',  ( -7.361458979222200050, -282.4271248920397284, -201.9875616782010184 ) ) ;
#74796=CARTESIAN_POINT ( 'NONE',  ( -67.32619353486499847, -294.9639438699124412, -337.0000461916976064 ) ) ;
#74798=CARTESIAN_POINT ( 'NONE',  ( -54.42813229853333468, -271.3380690714489560, -195.3538533559490702 ) ) ;
#74799=CARTESIAN_POINT ( 'NONE',  ( -106.6930801248616518, -272.1743473409617877, -237.2772108291333666 ) ) ;
#74800=CARTESIAN_POINT ( 'NONE',  ( 37.23513436521464826, -288.6517237077571281, -253.2269077795868384 ) ) ;
#74801=CARTESIAN_POINT ( 'NONE',  ( -68.75990146923227542, -289.3104004548721377, -336.2541876411106045 ) ) ;
#74802=CARTESIAN_POINT ( 'NONE',  ( -104.0052310366334467, -280.4941193760802776, -238.8296235851034339 ) ) ;
#74803=CARTESIAN_POINT ( 'NONE',  ( -55.56454454115822728, -299.5747044636771648, -198.5731343292042084 ) ) ;
#74805=CARTESIAN_POINT ( 'NONE',  ( -5.371745099425447201, -279.2774097796182105, -204.2925741684289278 ) ) ;
#74807=CARTESIAN_POINT ( 'NONE',  ( -60.13777720807046023, -297.4313900022854682, -196.7795409625197749 ) ) ;
#74808=CARTESIAN_POINT ( 'NONE',  ( 0.6228307675309368019, -294.4826844433272299, -206.3298085181062334 ) ) ;
#74811=CARTESIAN_POINT ( 'NONE',  ( -92.48315876940741020, -290.5195365815749255, -318.4295884558733292 ) ) ;
#74813=CARTESIAN_POINT ( 'NONE',  ( 32.20019090196863942, -291.3023189769452301, -240.2906861610345004 ) ) ;
#74814=CARTESIAN_POINT ( 'NONE',  ( -95.30326288283188774, -296.8437399085175343, -225.9274061157932749 ) ) ;
#74816=CARTESIAN_POINT ( 'NONE',  ( -113.1226066050086416, -291.9539293853587196, -279.7384554647178447 ) ) ;
#74817=CARTESIAN_POINT ( 'NONE',  ( -55.63300648810263738, -288.3376638359845288, -190.3683826091709363 ) ) ;
#74818=CARTESIAN_POINT ( 'NONE',  ( 36.08793221653890981, -289.7388097344805828, -284.8537513898409088 ) ) ;
#74819=CARTESIAN_POINT ( 'NONE',  ( 8.688526206528544904, -274.4199449389277561, -329.4292201027177498 ) ) ;
#74820=CARTESIAN_POINT ( 'NONE',  ( 21.99936111227792424, -278.0916381359802472, -315.3050013448788604 ) ) ;
#74821=CARTESIAN_POINT ( 'NONE',  ( -52.64232983163152824, -289.9345947764307425, -197.4576314366296685 ) ) ;
#74822=CARTESIAN_POINT ( 'NONE',  ( -70.71224548923348152, -281.4771313512563324, -202.3411783547301468 ) ) ;
#74826=CARTESIAN_POINT ( 'NONE',  ( 33.74733140475464666, -281.1258653181992599, -287.4508461675712852 ) ) ;
#74827=CARTESIAN_POINT ( 'NONE',  ( -110.2600863869629535, -279.9337980626911531, -246.4353390318107131 ) ) ;
#74829=CARTESIAN_POINT ( 'NONE',  ( -71.57513316140291693, -282.2892814199485088, -338.8890741972012393 ) ) ;
#74831=CARTESIAN_POINT ( 'NONE',  ( -56.85261729625045746, -278.2389087233992200, -344.6598165695388616 ) ) ;
#74833=CARTESIAN_POINT ( 'NONE',  ( -57.95311786317303415, -275.3108673175764238, -196.8359410454326337 ) ) ;
#74834=CARTESIAN_POINT ( 'NONE',  ( 17.40634833298267736, -278.6948066931273047, -313.9805196606274080 ) ) ;
#74836=CARTESIAN_POINT ( 'NONE',  ( -110.2370219626862422, -298.3250803578176260, -288.0581237040789802 ) ) ;
#74837=CARTESIAN_POINT ( 'NONE',  ( -108.6478968032355965, -291.4082403328366695, -287.3802951183754431 ) ) ;
#74838=CARTESIAN_POINT ( 'NONE',  ( -9.907990234155761300, -290.4588826358656775, -341.2227124832272693 ) ) ;
#74839=CARTESIAN_POINT ( 'NONE',  ( -99.79439238707358584, -290.4232890279208732, -232.3669882039579591 ) ) ;
#74840=CARTESIAN_POINT ( 'NONE',  ( 33.80491605301907754, -286.6857798815771616, -240.9356325364724398 ) ) ;
#74842=CARTESIAN_POINT ( 'NONE',  ( -68.13656191716009403, -281.8633256563235818, -337.4291200749680684 ) ) ;
#74843=CARTESIAN_POINT ( 'NONE',  ( 35.74182787285965190, -289.5815393327949323, -283.3866090234290596 ) ) ;
#74844=CARTESIAN_POINT ( 'NONE',  ( -111.0843622249936260, -283.0250433613940118, -270.8951863274088510 ) ) ;
#74845=CARTESIAN_POINT ( 'NONE',  ( 34.42558532079772959, -283.0747971231998008, -286.1946336673440214 ) ) ;
#74846=CARTESIAN_POINT ( 'NONE',  ( 39.40455292340610782, -288.4722885280886544, -268.6780092973235696 ) ) ;
#74847=CARTESIAN_POINT ( 'NONE',  ( -106.5050140291096881, -279.3590035408768699, -246.6594963076486806 ) ) ;
#74848=CARTESIAN_POINT ( 'NONE',  ( 29.13869172682219855, -291.8500721272266674, -232.3037111278238456 ) ) ;
#74850=CARTESIAN_POINT ( 'NONE',  ( 37.86334881235956829, -288.1566751647874867, -254.5380263817201296 ) ) ;
#74851=CARTESIAN_POINT ( 'NONE',  ( -65.86038291797562749, -286.1812710007635019, -198.8892129976321996 ) ) ;
#74852=CARTESIAN_POINT ( 'NONE',  ( -48.32658831639685815, -283.3625489863810003, -342.5298940285710501 ) ) ;
#74855=CARTESIAN_POINT ( 'NONE',  ( 29.79325560629463610, -294.9507952855915391, -235.1312481009662179 ) ) ;
#74856=CARTESIAN_POINT ( 'NONE',  ( -4.728055235960237468, -293.3163640789113060, -339.5827794190420832 ) ) ;
#74857=CARTESIAN_POINT ( 'NONE',  ( -66.90861186545470218, -276.5081731141227692, -337.3626566141915646 ) ) ;
#74858=CARTESIAN_POINT ( 'NONE',  ( -103.7575757838931594, -296.4069320112704418, -231.4974030807680379 ) ) ;
#74859=CARTESIAN_POINT ( 'NONE',  ( 18.48512608122216605, -292.7108980287340501, -318.4851670833149342 ) ) ;
#74860=CARTESIAN_POINT ( 'NONE',  ( -70.90734541729170815, -295.8429429994072848, -204.3824678880895078 ) ) ;
#74861=CARTESIAN_POINT ( 'NONE',  ( -34.85914000030421533, -293.2891090850193905, -197.0060404420374311 ) ) ;
#74862=CARTESIAN_POINT ( 'NONE',  ( 13.10595554735863111, -293.8571499198620813, -217.1703282730994147 ) ) ;
#74864=CARTESIAN_POINT ( 'NONE',  ( 21.71506595407890572, -292.1892730876040787, -316.8825864470006763 ) ) ;
#74865=CARTESIAN_POINT ( 'NONE',  ( -70.50246868630219410, -299.6151596358483289, -203.0762973128101692 ) ) ;
#74866=CARTESIAN_POINT ( 'NONE',  ( 34.51735257475012730, -288.6800724584279010, -284.5569920796708061 ) ) ;
#74869=CARTESIAN_POINT ( 'NONE',  ( -31.55095382332170217, -278.9594100142318780, -345.5449938028233419 ) ) ;
#74870=CARTESIAN_POINT ( 'NONE',  ( -75.15362639801952582, -276.3394030888983366, -336.9814373344150908 ) ) ;
#74871=CARTESIAN_POINT ( 'NONE',  ( -63.51459467862234476, -273.0684028178719700, -198.0541862448038728 ) ) ;
#74872=CARTESIAN_POINT ( 'NONE',  ( 36.95863206861560712, -279.5730284614820675, -265.8031764568244739 ) ) ;
#74873=CARTESIAN_POINT ( 'NONE',  ( -3.103020481910842676, -275.0073822010312483, -338.4502570589072548 ) ) ;
#74874=CARTESIAN_POINT ( 'NONE',  ( -100.5994214164760621, -294.7251764882240650, -307.8739816794015383 ) ) ;
#74875=CARTESIAN_POINT ( 'NONE',  ( -82.73167276013245441, -275.4322983545054058, -210.5910720037404644 ) ) ;
#74876=CARTESIAN_POINT ( 'NONE',  ( -89.32047147676225052, -273.9475478392272407, -218.9597561601831046 ) ) ;
#74878=CARTESIAN_POINT ( 'NONE',  ( -111.5478211001983340, -288.7397928283889428, -257.2516399299115051 ) ) ;
#74879=CARTESIAN_POINT ( 'NONE',  ( 23.79465795860887667, -274.8326992061354304, -230.4694431067368612 ) ) ;
#74880=CARTESIAN_POINT ( 'NONE',  ( 38.78557269228230098, -287.4064779481510641, -258.7131255145027922 ) ) ;
#74881=CARTESIAN_POINT ( 'NONE',  ( 73.34442978824353077, -301.4111611709244585, -194.9687698576807122 ) ) ;
#74882=CARTESIAN_POINT ( 'NONE',  ( -70.56022795400670589, -293.4910443592804654, -337.4174960522173023 ) ) ;
#74883=CARTESIAN_POINT ( 'NONE',  ( -102.7859114191754202, -283.2219714936363744, -310.6254201458635293 ) ) ;
#74885=CARTESIAN_POINT ( 'NONE',  ( -36.57589803479088175, -281.0423852956001269, -345.3697597730645725 ) ) ;
#74887=CARTESIAN_POINT ( 'NONE',  ( -91.03927565630729646, -290.0628654286411461, -220.3055446783482978 ) ) ;
#74888=CARTESIAN_POINT ( 'NONE',  ( -95.26341025021616815, -282.0463312047815521, -316.8134598304931160 ) ) ;
#74891=CARTESIAN_POINT ( 'NONE',  ( -110.3017899708364524, -288.3289069932375241, -287.7342565381404711 ) ) ;
#74892=CARTESIAN_POINT ( 'NONE',  ( -8.719245150118359433, -275.9535910364672304, -202.3989496974445785 ) ) ;
#74893=CARTESIAN_POINT ( 'NONE',  ( 1.903954844057003548, -283.7442703260256849, -336.1470380886358953 ) ) ;
#74894=CARTESIAN_POINT ( 'NONE',  ( -60.40782733873081156, -271.8353223806120695, -198.3533003457394557 ) ) ;
#74895=CARTESIAN_POINT ( 'NONE',  ( -110.3904209699347660, -284.5449207452787164, -270.9092993435457402 ) ) ;
#74896=CARTESIAN_POINT ( 'NONE',  ( -6.009396192098829914, -278.0573377870063609, -336.9607461438483824 ) ) ;
#74897=CARTESIAN_POINT ( 'NONE',  ( 33.40093977656022162, -276.6007997695163567, -289.0180369859816665 ) ) ;
#74898=CARTESIAN_POINT ( 'NONE',  ( -67.06469123073790684, -285.4419288368255820, -339.2199914195545603 ) ) ;
#74901=CARTESIAN_POINT ( 'NONE',  ( 24.02769098527455682, -294.0050566045246114, -316.8670083503797059 ) ) ;
#74902=CARTESIAN_POINT ( 'NONE',  ( -16.74161553446928252, -288.2993147639137987, -198.5611211504140954 ) ) ;
#74903=FACE_BOUND ( 'NONE', #88091, .T. ) ;
#74904=CARTESIAN_POINT ( 'NONE',  ( -111.2586520408596868, -288.4809262143061801, -234.7283546768995564 ) ) ;
#74905=CARTESIAN_POINT ( 'NONE',  ( -104.5161868564779297, -277.9536784139929750, -233.3600255426135277 ) ) ;
#74906=CARTESIAN_POINT ( 'NONE',  ( -92.22162211281154498, -289.6840599446832698, -217.4217697551215736 ) ) ;
#74907=CARTESIAN_POINT ( 'NONE',  ( -110.3013599312360213, -286.2078269172327509, -259.9882787384710241 ) ) ;
#74909=CARTESIAN_POINT ( 'NONE',  ( -54.16274406257657859, -279.0311278926650971, -342.4905113027081711 ) ) ;
#74910=CARTESIAN_POINT ( 'NONE',  ( -23.90747783461152309, -287.6456743716511824, -195.0867894278129029 ) ) ;
#74911=CARTESIAN_POINT ( 'NONE',  ( 33.24534612874339246, -283.8826458225866531, -295.8618016302511364 ) ) ;
#74912=CARTESIAN_POINT ( 'NONE',  ( 36.06327344518754074, -276.0110979503392628, -293.6142867819698949 ) ) ;
#74913=CARTESIAN_POINT ( 'NONE',  ( -93.05613846764882169, -295.2670227711166149, -220.6846832803128109 ) ) ;
#74914=CARTESIAN_POINT ( 'NONE',  ( -114.0436957555450022, -278.4773857616074793, -263.0118140440122261 ) ) ;
#74915=CARTESIAN_POINT ( 'NONE',  ( -50.22674051544231588, -299.8065700181458055, -197.0447492133035894 ) ) ;
#74918=CARTESIAN_POINT ( 'NONE',  ( -9.648957191793451571, -296.5349061383343496, -194.6049747682645545 ) ) ;
#74920=CARTESIAN_POINT ( 'NONE',  ( -108.2333168800458196, -277.8261538134307216, -288.0866214686623721 ) ) ;
#74921=CARTESIAN_POINT ( 'NONE',  ( -32.72196284039141290, -275.3141968799232586, -193.8845356672919706 ) ) ;
#74922=CARTESIAN_POINT ( 'NONE',  ( 39.38425109435739557, -280.6414980313104479, -272.8000975467962235 ) ) ;
#74923=CARTESIAN_POINT ( 'NONE',  ( 26.58240732987940191, -289.8185032158293666, -307.7677501940842717 ) ) ;
#74924=CARTESIAN_POINT ( 'NONE',  ( -67.93031800254712493, -296.9665896641506038, -340.2685153787912213 ) ) ;
#74925=CARTESIAN_POINT ( 'NONE',  ( -86.13055729043941255, -296.9167229438172058, -329.4174989609309137 ) ) ;
#74926=CARTESIAN_POINT ( 'NONE',  ( 21.61183459743630664, -294.9182611419863065, -224.2479829775269309 ) ) ;
#74927=CARTESIAN_POINT ( 'NONE',  ( 17.14364192129744069, -280.2731301447624332, -321.7327876833887785 ) ) ;
#74928=CARTESIAN_POINT ( 'NONE',  ( -32.90107183015801695, -282.0286959102318747, -196.0536821543844326 ) ) ;
#74929=CARTESIAN_POINT ( 'NONE',  ( -106.0827918770839062, -295.0076637180445687, -241.7958155944000680 ) ) ;
#74930=CARTESIAN_POINT ( 'NONE',  ( -103.7101143763073594, -285.6601231016950351, -307.9068764114813916 ) ) ;
#74932=CARTESIAN_POINT ( 'NONE',  ( 25.22165381111244642, -285.9482554238093144, -232.1504804965943265 ) ) ;
#74933=CARTESIAN_POINT ( 'NONE',  ( 38.04397856571704040, -281.0907911423005885, -285.5371594570767684 ) ) ;
#74934=CARTESIAN_POINT ( 'NONE',  ( 199.0721941440129115, 283.7445530891940280, -111.5641654068537463 ) ) ;
#74936=CARTESIAN_POINT ( 'NONE',  ( -48.79871030906058138, -287.7699243380597522, -345.9616115326194858 ) ) ;
#74937=CARTESIAN_POINT ( 'NONE',  ( -12.01066960404757999, -286.0578619286990829, -201.8744303757225964 ) ) ;
#74939=CARTESIAN_POINT ( 'NONE',  ( -94.16085711432764072, -284.9290770016187366, -321.8886088185550989 ) ) ;
#74940=CARTESIAN_POINT ( 'NONE',  ( 34.39347784178688983, -275.7055030471343002, -256.7173747838750728 ) ) ;
#74941=CARTESIAN_POINT ( 'NONE',  ( -68.19175489789289202, -290.5767579684503517, -200.1345132356656791 ) ) ;
#74942=CARTESIAN_POINT ( 'NONE',  ( 23.32761967868425046, -282.8358363006686886, -317.6322293528140221 ) ) ;
#74944=CARTESIAN_POINT ( 'NONE',  ( -53.63151622411897534, -281.3670620229088399, -195.7594043319838875 ) ) ;
#74945=CARTESIAN_POINT ( 'NONE',  ( 37.96309648552013272, -281.6849037842736720, -254.3314863607673431 ) ) ;
#74946=CARTESIAN_POINT ( 'NONE',  ( -67.68488546085839630, -289.1237833571631768, -207.2794874003663779 ) ) ;
#74947=CARTESIAN_POINT ( 'NONE',  ( 65.37179972839517461, 47.69369081529824683, -319.0422732978356635 ) ) ;
#74949=CARTESIAN_POINT ( 'NONE',  ( 35.37389569884855689, -277.7804538021955523, -288.0920117263862039 ) ) ;
#74950=CARTESIAN_POINT ( 'NONE',  ( -96.18930935400858573, -239.3917820358037147, -341.2764046406296075 ) ) ;
#74951=CARTESIAN_POINT ( 'NONE',  ( -2.356358904441790969, -278.5374919569934491, -204.4082177598831151 ) ) ;
#74952=CARTESIAN_POINT ( 'NONE',  ( -68.08283579577219768, -296.9861272120068065, -204.0234178517839609 ) ) ;
#74953=CARTESIAN_POINT ( 'NONE',  ( 29.51808526316253278, -293.5558047644756812, -308.5383472440107653 ) ) ;
#74955=CARTESIAN_POINT ( 'NONE',  ( -36.53001837626698034, -296.6368610634120841, -193.9505346561512908 ) ) ;
#74956=CARTESIAN_POINT ( 'NONE',  ( -93.02865121654770064, -288.2683587841124222, -318.8668834992717507 ) ) ;
#74957=CARTESIAN_POINT ( 'NONE',  ( -72.69225968962392415, -297.3858689795047781, -335.6535200827408971 ) ) ;
#74958=CARTESIAN_POINT ( 'NONE',  ( 2.701783047342122934, -287.9169486293366162, -208.7351256373478350 ) ) ;
#74960=CARTESIAN_POINT ( 'NONE',  ( 20.19436347908770557, -293.8029380839086002, -219.5237299995925468 ) ) ;
#74961=CARTESIAN_POINT ( 'NONE',  ( -107.0426873680625732, -284.7544289292448525, -292.2645610786594261 ) ) ;
#74962=CARTESIAN_POINT ( 'NONE',  ( -36.53035058957745207, -296.8570283620464920, -193.7583493993183197 ) ) ;
#74963=CARTESIAN_POINT ( 'NONE',  ( -2.138946065623450465, -293.3089572078238803, -202.0461164777274519 ) ) ;
#74964=CARTESIAN_POINT ( 'NONE',  ( -88.61314469272407734, -291.8475827130143330, -212.9959205599886900 ) ) ;
#74965=CARTESIAN_POINT ( 'NONE',  ( -75.86693808531906313, -289.7490311545278132, -332.3676180034215690 ) ) ;
#74967=CARTESIAN_POINT ( 'NONE',  ( -98.93149485913795615, -299.0067802050005525, -226.2362648170815476 ) ) ;
#74968=CARTESIAN_POINT ( 'NONE',  ( -95.71509681338280018, -272.0194528579862094, -220.7369422418896363 ) ) ;
#74969=CARTESIAN_POINT ( 'NONE',  ( 15.98900708128109294, -281.3318678153616474, -320.6263401596224867 ) ) ;
#74972=CARTESIAN_POINT ( 'NONE',  ( -96.10624957826553327, -277.3900087657607969, -320.0428544424643746 ) ) ;
#74973=CARTESIAN_POINT ( 'NONE',  ( -81.53393939933268086, -271.8397045178370490, -211.1912845992768268 ) ) ;
#74974=CARTESIAN_POINT ( 'NONE',  ( -105.3943992517899204, -280.0188803207770434, -300.1494931195694562 ) ) ;
#74975=CARTESIAN_POINT ( 'NONE',  ( -43.32995393014883945, -275.2681635241457343, -344.3544034679648007 ) ) ;
#74976=CARTESIAN_POINT ( 'NONE',  ( -109.2707992808299480, -297.5647754325951837, -285.0296439101198303 ) ) ;
#74977=CARTESIAN_POINT ( 'NONE',  ( -43.51386669990820621, -274.9136702676119626, -197.3355026116745137 ) ) ;
#74978=CARTESIAN_POINT ( 'NONE',  ( -89.08022788900238709, -298.9395783275885492, -214.3471053572679352 ) ) ;
#74979=CARTESIAN_POINT ( 'NONE',  ( -49.42999155827750002, -271.9190247064548203, -195.9291656270295618 ) ) ;
#74980=CARTESIAN_POINT ( 'NONE',  ( 24.93035956269229914, -293.6753372697427267, -231.9755710365363086 ) ) ;
#74981=CARTESIAN_POINT ( 'NONE',  ( 34.22502406583749490, -291.9020001822214567, -253.1730831051700079 ) ) ;
#74983=CARTESIAN_POINT ( 'NONE',  ( -82.50508948364219464, -278.1432255321193452, -332.6491197564680533 ) ) ;
#74985=CARTESIAN_POINT ( 'NONE',  ( -55.30296780347217833, -298.1480740145520372, -199.5311087887484405 ) ) ;
#74987=CARTESIAN_POINT ( 'NONE',  ( 19.40639413506759325, -280.9389721845145687, -321.7509049821683789 ) ) ;
#74988=CARTESIAN_POINT ( 'NONE',  ( 19.98632690472514639, -296.2235695314948885, -318.9772238127679316 ) ) ;
#74990=CARTESIAN_POINT ( 'NONE',  ( -53.73577489193964851, -282.4649882219028427, -341.7143434471876162 ) ) ;
#74991=CARTESIAN_POINT ( 'NONE',  ( -65.90378027287727036, -281.4247720116724736, -339.9036388608907373 ) ) ;
#74992=CARTESIAN_POINT ( 'NONE',  ( 24.29687438552565482, -273.5743099281897912, -230.1608561809034654 ) ) ;
#74993=CARTESIAN_POINT ( 'NONE',  ( 35.64905448056661896, -283.7743637483688985, -287.6596787865418037 ) ) ;
#74996=CARTESIAN_POINT ( 'NONE',  ( -10.60898051455994029, -272.7948574946798317, -198.9481130326471998 ) ) ;
#74997=CARTESIAN_POINT ( 'NONE',  ( -91.98333423252027785, -279.8295787475494762, -322.0528317694735279 ) ) ;
#74999=CARTESIAN_POINT ( 'NONE',  ( 11.13464723912138155, -288.6370904760748886, -212.3328932701232361 ) ) ;
#75001=CARTESIAN_POINT ( 'NONE',  ( -110.9014145276504166, -288.3633514973482193, -285.0530060899549198 ) ) ;
#75003=CARTESIAN_POINT ( 'NONE',  ( -110.7711711056071806, -295.3687492845581346, -268.7087269803420213 ) ) ;
#75004=CARTESIAN_POINT ( 'NONE',  ( -81.15530590461534644, -287.7937389005547857, -330.3519999747874749 ) ) ;
#75005=CARTESIAN_POINT ( 'NONE',  ( -110.2140130185358942, -271.2396475792842807, -270.3444066551136871 ) ) ;
#75006=CARTESIAN_POINT ( 'NONE',  ( -106.8240884546824105, -294.1838755858004220, -298.5958193036719308 ) ) ;
#75007=CARTESIAN_POINT ( 'NONE',  ( -7.211669185547437522, -287.1439547021541330, -340.4814972528461112 ) ) ;
#75008=CARTESIAN_POINT ( 'NONE',  ( 21.95978501899401891, -282.5427527767596985, -226.4106600185252205 ) ) ;
#75009=CARTESIAN_POINT ( 'NONE',  ( -55.48227051209320848, -281.5223412516061785, -344.1506410698469836 ) ) ;
#75010=CARTESIAN_POINT ( 'NONE',  ( -60.25896621304476497, -291.7467374322102387, -200.9986347882887685 ) ) ;
#75011=CARTESIAN_POINT ( 'NONE',  ( 30.55824450589305030, -282.5998743493864822, -241.9890818482705583 ) ) ;
#75012=CARTESIAN_POINT ( 'NONE',  ( 10.02099698800581429, -283.1828960342839423, -326.1895338140733998 ) ) ;
#75013=CARTESIAN_POINT ( 'NONE',  ( 37.93307386394651814, -289.4749126423944290, -265.8903018629110306 ) ) ;
#75014=CARTESIAN_POINT ( 'NONE',  ( -46.13197965235344356, -298.1102525112013950, -193.8645102774957252 ) ) ;
#75015=CARTESIAN_POINT ( 'NONE',  ( 21.73062588760889469, -276.2168232603145270, -319.7520108586359129 ) ) ;
#75016=CARTESIAN_POINT ( 'NONE',  ( -32.06563897406375929, -294.0989051586685719, -195.8901044153024031 ) ) ;
#75018=CARTESIAN_POINT ( 'NONE',  ( -54.42813229853333468, -285.7662352645560873, -345.3683826091709648 ) ) ;
#75019=CARTESIAN_POINT ( 'NONE',  ( 26.08775556333124257, -274.0946431784811921, -310.7905922601033240 ) ) ;
#75021=CARTESIAN_POINT ( 'NONE',  ( -72.88909305817860229, -295.9894778522260026, -202.9024242050108455 ) ) ;
#75022=CARTESIAN_POINT ( 'NONE',  ( -109.4399411817046399, -291.9459649576813831, -286.1768208103741244 ) ) ;
#75023=CARTESIAN_POINT ( 'NONE',  ( -4.050869510497753900, -273.8518091038874331, -205.2654755580136339 ) ) ;
#75024=CARTESIAN_POINT ( 'NONE',  ( -94.84395932248192196, -292.7176838635762124, -224.2520377888179439 ) ) ;
#75025=CARTESIAN_POINT ( 'NONE',  ( -101.3350937672449561, -291.9800218234397562, -234.6443747098917925 ) ) ;
#75026=CARTESIAN_POINT ( 'NONE',  ( -109.7061544568813076, -286.1093759542301882, -285.9569864571572566 ) ) ;
#75027=CARTESIAN_POINT ( 'NONE',  ( -113.5234499958223893, -291.8947469192067388, -276.9212109880714934 ) ) ;
#75028=CARTESIAN_POINT ( 'NONE',  ( -44.86532644363411038, -293.2741064018957218, -194.1725158200438273 ) ) ;
#75029=CARTESIAN_POINT ( 'NONE',  ( 30.58478177080551319, -293.7447035494981833, -297.2387664234243516 ) ) ;
#75030=CARTESIAN_POINT ( 'NONE',  ( 37.68025710328415556, -289.5249655824406432, -268.2309175286733876 ) ) ;
#75031=CARTESIAN_POINT ( 'NONE',  ( 32.02054409016238878, -281.2885222562746321, -236.8037600104784701 ) ) ;
#75032=CARTESIAN_POINT ( 'NONE',  ( -37.23068762374366969, -296.1333855492536600, -194.8003966492061068 ) ) ;
#75033=CARTESIAN_POINT ( 'NONE',  ( -68.49881234312341860, -285.4872935870988613, -199.9320107437874583 ) ) ;
#75034=CARTESIAN_POINT ( 'NONE',  ( 35.98463295030797582, -277.3518478826539422, -256.3934523764798996 ) ) ;
#75035=CARTESIAN_POINT ( 'NONE',  ( -71.60778444644189733, -282.3104605907287237, -335.2684825200851151 ) ) ;
#75036=CARTESIAN_POINT ( 'NONE',  ( -5.596708187631768361, -284.4695189655774357, -202.4107232842063411 ) ) ;
#75037=CARTESIAN_POINT ( 'NONE',  ( -110.9803579279968062, -276.4645190657357716, -288.2383647405698071 ) ) ;
#75039=CARTESIAN_POINT ( 'NONE',  ( -82.83793702502916290, -283.2011666578981703, -327.5931726714594561 ) ) ;
#75040=CARTESIAN_POINT ( 'NONE',  ( -36.77100394507235848, -281.2642460662276562, -193.7473369856338934 ) ) ;
#75041=CARTESIAN_POINT ( 'NONE',  ( 37.87533220225556363, -286.8033008045121051, -285.6979449421966137 ) ) ;
#75042=CARTESIAN_POINT ( 'NONE',  ( 36.21661521024648778, -295.4247907433466480, -279.0069592076075651 ) ) ;
#75043=CARTESIAN_POINT ( 'NONE',  ( 15.45788751321450682, -276.3839091825635705, -215.4189305574670357 ) ) ;
#75044=CARTESIAN_POINT ( 'NONE',  ( -13.23385828139068465, -275.6740776308764111, -197.7518194496450405 ) ) ;
#75045=CARTESIAN_POINT ( 'NONE',  ( -69.25333309265458581, -277.3173327406349244, -336.0304780688007327 ) ) ;
#75046=CARTESIAN_POINT ( 'NONE',  ( -97.62429825329751054, -275.1358554311934199, -226.2541291272155206 ) ) ;
#75047=CARTESIAN_POINT ( 'NONE',  ( 35.79720624615365665, -285.7564829527370307, -286.2555383435764611 ) ) ;
#75049=CARTESIAN_POINT ( 'NONE',  ( -113.2123576640155846, -292.2486240136522611, -262.7374718060261785 ) ) ;
#75050=CARTESIAN_POINT ( 'NONE',  ( 35.84421031392759005, -292.4061056126957396, -265.3086779758943976 ) ) ;
#75052=CARTESIAN_POINT ( 'NONE',  ( 27.50726076503848816, -292.7625326869556943, -236.7947693910804503 ) ) ;
#75054=CARTESIAN_POINT ( 'NONE',  ( 5.396507794224528531, -289.5679308636480869, -334.0395137907563026 ) ) ;
#75055=CARTESIAN_POINT ( 'NONE',  ( -22.18135550578324455, -280.9027802450719378, -198.7965567756323821 ) ) ;
#75056=CARTESIAN_POINT ( 'NONE',  ( -87.25062962735587746, -296.2960774483836985, -212.0623382339854857 ) ) ;
#75057=CARTESIAN_POINT ( 'NONE',  ( 12.00580347735084530, -287.3685537827529402, -211.3159110462754313 ) ) ;
#75058=CARTESIAN_POINT ( 'NONE',  ( 22.07114813388301400, -287.2276021418553000, -221.4136180153494990 ) ) ;
#75059=CARTESIAN_POINT ( 'NONE',  ( -107.3764512311631307, -285.1609418250956196, -249.5163859517256526 ) ) ;
#75060=CARTESIAN_POINT ( 'NONE',  ( -48.42808399934508401, -154.7767485661955220, -365.1229883189888596 ) ) ;
#75061=CARTESIAN_POINT ( 'NONE',  ( 200.1221584904331792, 292.9742979738146005, -82.85065899227846842 ) ) ;
#75062=CARTESIAN_POINT ( 'NONE',  ( 84.11129044875666239, 81.79000652128765125, -298.7613687047784765 ) ) ;
#75063=CARTESIAN_POINT ( 'NONE',  ( 3.215143990356036152, -275.6888087619737462, -331.2523663012747193 ) ) ;
#75064=CARTESIAN_POINT ( 'NONE',  ( -97.14579705661100206, -276.8826996728543577, -312.7821710251181457 ) ) ;
#75065=CARTESIAN_POINT ( 'NONE',  ( -33.33216815981333525, -297.6087474355353493, -193.4229804999733346 ) ) ;
#75066=CARTESIAN_POINT ( 'NONE',  ( -75.59557456435523193, -208.9939761195755921, -354.3369844704666889 ) ) ;
#75067=CARTESIAN_POINT ( 'NONE',  ( -25.86060984566115195, -275.5936643199162859, -346.0016021008059965 ) ) ;
#75068=CARTESIAN_POINT ( 'NONE',  ( -68.77878093516920899, -289.9693209652417636, -336.3133612515398454 ) ) ;
#75069=CARTESIAN_POINT ( 'NONE',  ( -31.93394254334309323, -298.9210700721320109, -193.5218773760562385 ) ) ;
#75070=CARTESIAN_POINT ( 'NONE',  ( -114.0799253280429895, -273.2751830130413850, -264.6420974808686992 ) ) ;
#75071=CARTESIAN_POINT ( 'NONE',  ( -38.34016387664090786, -295.2316939061437324, -343.3542894075472418 ) ) ;
#75073=CARTESIAN_POINT ( 'NONE',  ( -20.42426950876691549, -278.7568184255255233, -344.0566180169374775 ) ) ;
#75075=CARTESIAN_POINT ( 'NONE',  ( 35.54876346154662770, -281.3721211855328761, -295.1540119256617913 ) ) ;
#75076=CARTESIAN_POINT ( 'NONE',  ( -109.3442982440810880, -279.4499591290078797, -284.2060585748386075 ) ) ;
#75077=CARTESIAN_POINT ( 'NONE',  ( -31.50543159089326650, -278.7396945082627440, -346.1752553180350560 ) ) ;
#75078=CARTESIAN_POINT ( 'NONE',  ( -100.3923504785746843, -295.6460241302178815, -232.3148560197450934 ) ) ;
#75081=CARTESIAN_POINT ( 'NONE',  ( -105.2670220793525004, -278.3612027709063454, -297.1034185998467478 ) ) ;
#75082=CARTESIAN_POINT ( 'NONE',  ( -21.39829406683040247, -275.0544505095984960, -195.1948581104310563 ) ) ;
#75083=CARTESIAN_POINT ( 'NONE',  ( 35.47323088189300222, -286.5341576688471150, -293.8405578095191117 ) ) ;
#75084=CARTESIAN_POINT ( 'NONE',  ( 12.61287353947355960, -276.7482455577631981, -214.3494362579301935 ) ) ;
#75085=CARTESIAN_POINT ( 'NONE',  ( 12.30788512090503417, -274.9512057929173920, -328.4431718026235103 ) ) ;
#75087=CARTESIAN_POINT ( 'NONE',  ( -68.83673463839879503, -288.6743509334596069, -336.3964458666311543 ) ) ;
#75089=CARTESIAN_POINT ( 'NONE',  ( -78.46094456981056453, -284.8626585114653835, -205.3801936818713614 ) ) ;
#75090=CARTESIAN_POINT ( 'NONE',  ( -4.395952960888336314, -280.8516643341324084, -336.6374467878439987 ) ) ;
#75091=CARTESIAN_POINT ( 'NONE',  ( 33.88931698763983036, -280.3694859963403587, -288.8914438805327904 ) ) ;
#75092=CARTESIAN_POINT ( 'NONE',  ( -86.66229079310933514, -283.4405736102248170, -214.5356880583871657 ) ) ;
#75093=CARTESIAN_POINT ( 'NONE',  ( 17.52777596615658595, -290.2681200034230642, -321.5104330038002445 ) ) ;
#75094=CARTESIAN_POINT ( 'NONE',  ( -24.82367629390176234, -281.4204964335653472, -198.0394090487811241 ) ) ;
#75095=CARTESIAN_POINT ( 'NONE',  ( 197.0526033736561260, 285.3763917366303531, -111.7597979621280189 ) ) ;
#75096=CARTESIAN_POINT ( 'NONE',  ( -13.68979532640991437, -281.1500305604588448, -342.7974887736113487 ) ) ;
#75097=CARTESIAN_POINT ( 'NONE',  ( 27.84919351127164688, -296.0479111339789711, -307.5490808290019800 ) ) ;
#75098=CARTESIAN_POINT ( 'NONE',  ( -58.99169560465021789, -278.0156349317891227, -197.5239591445619283 ) ) ;
#75099=CARTESIAN_POINT ( 'NONE',  ( -73.37420219773780161, -285.5286868711398824, -336.3865040498762369 ) ) ;
#75101=CARTESIAN_POINT ( 'NONE',  ( -11.66600671786804888, -294.3039262087660290, -199.2422707158225705 ) ) ;
#75102=CARTESIAN_POINT ( 'NONE',  ( -7.978507348678490096, -274.6673593749728752, -339.3880970375254265 ) ) ;
#75103=CARTESIAN_POINT ( 'NONE',  ( 38.13349909226820955, -286.5687254150570880, -255.9509436752776992 ) ) ;
#75104=CARTESIAN_POINT ( 'NONE',  ( -70.56278798530524909, -290.0063903003613746, -204.4611958364363602 ) ) ;
#75106=CARTESIAN_POINT ( 'NONE',  ( -36.47706440237539738, -275.7259521424711579, -343.8617359984473865 ) ) ;
#75107=CARTESIAN_POINT ( 'NONE',  ( -5.024846877644730370, -292.7616979509086832, -337.2069370877067627 ) ) ;
#75108=CARTESIAN_POINT ( 'NONE',  ( -110.2768796039921568, -291.7488928151328196, -279.4000931797045837 ) ) ;
#75111=CARTESIAN_POINT ( 'NONE',  ( -1.115791215868618069, -291.0038824809078051, -203.2016713106322356 ) ) ;
#75112=CARTESIAN_POINT ( 'NONE',  ( -92.12865823314830038, -286.8533822087449039, -220.8407847019724954 ) ) ;
#75113=CARTESIAN_POINT ( 'NONE',  ( -86.74287878492778248, -287.9675926800250068, -328.1666967194076960 ) ) ;
#75114=CARTESIAN_POINT ( 'NONE',  ( 36.21983522669755473, -289.0220297267323986, -273.7691624788020022 ) ) ;
#75116=CARTESIAN_POINT ( 'NONE',  ( 15.13822182214966716, -287.6195731863443825, -219.3860307436418680 ) ) ;
#75117=CARTESIAN_POINT ( 'NONE',  ( -8.983120647694706307, -296.6631289151063697, -340.2318574784262069 ) ) ;
#75119=CARTESIAN_POINT ( 'NONE',  ( 11.81098053230759604, -287.9221272078049765, -211.5379960580004877 ) ) ;
#75120=CARTESIAN_POINT ( 'NONE',  ( -37.15553436594755254, -275.1296553738495732, -345.9337066439591695 ) ) ;
#75121=CARTESIAN_POINT ( 'NONE',  ( -114.0576561173024430, -278.7982106933513364, -277.3333872815952077 ) ) ;
#75122=CARTESIAN_POINT ( 'NONE',  ( -7.541254893382253854, -280.0989923328306759, -199.3702183362086942 ) ) ;
#75123=CARTESIAN_POINT ( 'NONE',  ( -37.17059980140709996, -300.0342024511551244, -195.7133385678558284 ) ) ;
#75125=CARTESIAN_POINT ( 'NONE',  ( -37.25363422452094397, -284.0530614461757750, -195.3483864762255848 ) ) ;
#75127=CARTESIAN_POINT ( 'NONE',  ( -110.0930979341945317, -276.8841374057031999, -255.5291876289126947 ) ) ;
#75128=CARTESIAN_POINT ( 'NONE',  ( 1.047956534388809535, -280.5395511379381333, -334.7911956633159889 ) ) ;
#75130=CARTESIAN_POINT ( 'NONE',  ( 31.22371092281886007, -274.4673064654773498, -303.9700947675825660 ) ) ;
#75131=CARTESIAN_POINT ( 'NONE',  ( -105.4099573643679122, -298.4473858951712941, -242.1224900475620530 ) ) ;
#75132=CARTESIAN_POINT ( 'NONE',  ( -70.34958911028151363, -282.3973219750861290, -339.5995918340052526 ) ) ;
#75133=CARTESIAN_POINT ( 'NONE',  ( -109.0118782206890842, -297.6922083110581525, -255.2410904326320349 ) ) ;
#75134=CARTESIAN_POINT ( 'NONE',  ( -106.0776466100415263, -298.3015003357391493, -236.7654645040389312 ) ) ;
#75135=CARTESIAN_POINT ( 'NONE',  ( -36.73163066710183955, -273.7267430296075190, -197.3301036909300308 ) ) ;
#75136=CARTESIAN_POINT ( 'NONE',  ( 35.39169231792075720, -295.7873720920933351, -288.6601418791511264 ) ) ;
#75137=CARTESIAN_POINT ( 'NONE',  ( 37.82540773039051629, -287.9284466310153334, -287.1217955889143241 ) ) ;
#75138=CARTESIAN_POINT ( 'NONE',  ( -93.86797833422095039, -277.3243317398768113, -220.2203753507405679 ) ) ;
#75139=CARTESIAN_POINT ( 'NONE',  ( -108.7992501029185917, -290.0214358306701570, -299.0459320151213660 ) ) ;
#75140=CARTESIAN_POINT ( 'NONE',  ( 34.75120964406034574, -286.7803240818519726, -283.2460242351291981 ) ) ;
#75141=CARTESIAN_POINT ( 'NONE',  ( -30.84446364412297825, -290.1339811201954149, -195.5916829181566925 ) ) ;
#75143=CARTESIAN_POINT ( 'NONE',  ( 207.9738562182569979, 291.4636489450775798, -54.00000000000000711 ) ) ;
#75144=CARTESIAN_POINT ( 'NONE',  ( -21.12177084167196384, -288.3460269611088052, -341.5994667520130292 ) ) ;
#75146=CARTESIAN_POINT ( 'NONE',  ( -99.59061886654667717, -284.8949282948299242, -315.3708891146958422 ) ) ;
#75147=CARTESIAN_POINT ( 'NONE',  ( 39.37130992499004378, -292.6462375692264573, -273.1779070958779698 ) ) ;
#75148=CARTESIAN_POINT ( 'NONE',  ( 18.78690920761983207, -282.1545319301108066, -218.3719124981581956 ) ) ;
#75149=CARTESIAN_POINT ( 'NONE',  ( -97.53355314180242885, -283.8094717073392417, -311.7522583352538277 ) ) ;
#75150=CARTESIAN_POINT ( 'NONE',  ( -70.72904229054118730, -297.6238744718751832, -200.9760663984699818 ) ) ;
#75151=CARTESIAN_POINT ( 'NONE',  ( -40.81489845350044021, -275.3228678541352679, -196.9000451500173767 ) ) ;
#75152=CARTESIAN_POINT ( 'NONE',  ( -67.19934872118521696, -289.6788351480227561, -201.9479056206777159 ) ) ;
#75153=CARTESIAN_POINT ( 'NONE',  ( -32.65040574288002517, -272.9074813964646182, -197.1015287273976639 ) ) ;
#75156=CARTESIAN_POINT ( 'NONE',  ( -104.2974026483663295, -286.0390227736058932, -303.0101445029939100 ) ) ;
#75157=CARTESIAN_POINT ( 'NONE',  ( -4.621884663425820605, -295.7108218673145643, -339.7362274928041757 ) ) ;
#75158=CARTESIAN_POINT ( 'NONE',  ( -73.61340645483336687, -286.2085504889698200, -206.8780575459666409 ) ) ;
#75159=CARTESIAN_POINT ( 'NONE',  ( -48.47175576450237600, -276.2491390529971795, -346.3684008123586295 ) ) ;
#75160=CARTESIAN_POINT ( 'NONE',  ( -19.41859543215960926, -292.9281362805288040, -195.5261913122782857 ) ) ;
#75161=CARTESIAN_POINT ( 'NONE',  ( 17.47447081539952762, -284.9642408447560911, -217.9834899676512805 ) ) ;
#75162=CARTESIAN_POINT ( 'NONE',  ( -47.74473749351228236, -292.2567392274605140, -194.0346617641090461 ) ) ;
#75163=CARTESIAN_POINT ( 'NONE',  ( -109.1989692998816963, -290.7141853976572747, -283.3465080036577888 ) ) ;
#75166=CARTESIAN_POINT ( 'NONE',  ( 65.43520553966946807, 46.08562840962796514, -315.4480577230399376 ) ) ;
#75167=CARTESIAN_POINT ( 'NONE',  ( -75.77440977838452341, -287.0693869736280703, -204.3788351212604084 ) ) ;
#75168=CARTESIAN_POINT ( 'NONE',  ( -37.30987171927208834, -277.5523547857346784, -190.3611179825600175 ) ) ;
#75170=CARTESIAN_POINT ( 'NONE',  ( -82.99793080373400755, -282.6139369486199939, -327.7824756983355883 ) ) ;
#75171=CARTESIAN_POINT ( 'NONE',  ( -80.21793177351976567, -277.2819247761232191, -334.3578544847962917 ) ) ;
#75172=CARTESIAN_POINT ( 'NONE',  ( 27.15166740907138987, -284.0620442495107909, -308.4192565516710829 ) ) ;
#75173=CARTESIAN_POINT ( 'NONE',  ( -81.69423236938992261, -220.3794719950213903, -351.4091104718835936 ) ) ;
#75174=CARTESIAN_POINT ( 'NONE',  ( 11.10489089610397961, -280.9715107882265102, -329.5187785198529582 ) ) ;
#75175=CARTESIAN_POINT ( 'NONE',  ( -1.372143591914971816, -284.5513449184772412, -204.8964043238619297 ) ) ;
#75176=CARTESIAN_POINT ( 'NONE',  ( -34.82413875304405337, -299.8433936276347254, -194.3737023588105046 ) ) ;
#75177=CARTESIAN_POINT ( 'NONE',  ( -106.0429118097728889, -296.7118090073012127, -295.3721027996700172 ) ) ;
#75179=CARTESIAN_POINT ( 'NONE',  ( 34.43504269336288814, -292.0293064091196698, -254.5122796499099138 ) ) ;
#75180=CARTESIAN_POINT ( 'NONE',  ( -70.24985648337967348, -278.1258464599048352, -339.8763704906940006 ) ) ;
#75181=CARTESIAN_POINT ( 'NONE',  ( 22.28083267413327917, -274.9639657297968824, -228.2187767536633771 ) ) ;
#75182=CARTESIAN_POINT ( 'NONE',  ( 31.57145899864639915, -274.9076861586110567, -304.1342088131229957 ) ) ;
#75184=CARTESIAN_POINT ( 'NONE',  ( -49.99709029990158626, -271.8906435319648267, -196.3846513585159528 ) ) ;
#75185=CARTESIAN_POINT ( 'NONE',  ( -37.66810429572120711, -296.4813938062350758, -346.7841728759144075 ) ) ;
#75186=EDGE_CURVE ( 'NONE', #1315, #53167, #59008, .T. ) ;
#75189=CARTESIAN_POINT ( 'NONE',  ( -66.67066573470455637, -284.5252904046245703, -337.5613349114591983 ) ) ;
#75190=CARTESIAN_POINT ( 'NONE',  ( -21.90959676427218739, -284.6171576765306099, -344.7642375212583943 ) ) ;
#75191=CARTESIAN_POINT ( 'NONE',  ( -99.69193064015632899, -284.4270119998699897, -232.1026485640697956 ) ) ;
#75192=CARTESIAN_POINT ( 'NONE',  ( 16.16400927475245197, -274.6768332154045993, -321.1900416037742616 ) ) ;
#75193=CARTESIAN_POINT ( 'NONE',  ( -36.15034286070351044, -284.8974740403209012, -344.5867614710153362 ) ) ;
#75194=CARTESIAN_POINT ( 'NONE',  ( -43.28209599835645349, -275.6084025865883405, -343.8146369557525190 ) ) ;
#75195=CARTESIAN_POINT ( 'NONE',  ( 21.09159888046461973, -277.2512914091990410, -314.6304712809431408 ) ) ;
#75197=CARTESIAN_POINT ( 'NONE',  ( -112.5615815435449321, -279.5523904734822054, -254.6091494186943294 ) ) ;
#75198=CARTESIAN_POINT ( 'NONE',  ( 1.337606918146148072, -281.0463607288460821, -203.7915311398326708 ) ) ;
#75201=CARTESIAN_POINT ( 'NONE',  ( 33.68786813897401800, -289.0737900418604340, -243.9962566957020158 ) ) ;
#75202=CARTESIAN_POINT ( 'NONE',  ( -110.2610756439923989, -295.6631948843017881, -276.9039334352452784 ) ) ;
#75203=EDGE_CURVE ( 'NONE', #78913, #69774, #74132, .T. ) ;
#75204=CARTESIAN_POINT ( 'NONE',  ( -113.0701926592480930, -290.0680571836127797, -257.0004216787720566 ) ) ;
#75205=CARTESIAN_POINT ( 'NONE',  ( 0.7085943880477741930, -284.8064485845953300, -206.8179028991024779 ) ) ;
#75206=CARTESIAN_POINT ( 'NONE',  ( -33.18738715785291760, -284.6800714410216528, -196.8390201679295899 ) ) ;
#75207=CARTESIAN_POINT ( 'NONE',  ( -101.1893004257353965, -288.2838404942792181, -307.8981629085842542 ) ) ;
#75208=CARTESIAN_POINT ( 'NONE',  ( -96.90600122926278459, -286.3539326375493488, -227.4534901750206188 ) ) ;
#75209=CARTESIAN_POINT ( 'NONE',  ( -45.45914416374635181, -275.1547142853006562, -344.9722231697173243 ) ) ;
#75210=CARTESIAN_POINT ( 'NONE',  ( 20.86461581374804553, -286.6215580877141633, -319.5390114096213665 ) ) ;
#75211=CARTESIAN_POINT ( 'NONE',  ( 35.76426420316494159, -289.3365992337932084, -253.5555168046678034 ) ) ;
#75212=CARTESIAN_POINT ( 'NONE',  ( 36.49421464330887943, -285.3715910766461548, -256.2797075733649308 ) ) ;
#75214=CARTESIAN_POINT ( 'NONE',  ( -2.305587835448050793, -283.5177268165709279, -334.6862566555413991 ) ) ;
#75215=CARTESIAN_POINT ( 'NONE',  ( -86.17360724881899614, -291.7272892405834455, -327.5737827586361277 ) ) ;
#75216=CARTESIAN_POINT ( 'NONE',  ( 82.12901144365632433, -301.1131897426192268, -194.1079538098041724 ) ) ;
#75218=CARTESIAN_POINT ( 'NONE',  ( -106.4657733041606917, -298.8705224153829931, -239.7164733156501200 ) ) ;
#75219=CARTESIAN_POINT ( 'NONE',  ( 37.34647655466836369, -279.4572050383280839, -262.9791462903383490 ) ) ;
#75220=CARTESIAN_POINT ( 'NONE',  ( -19.41450350732463903, -291.4741245015094933, -195.5884428077315818 ) ) ;
#75221=CARTESIAN_POINT ( 'NONE',  ( -101.9046953734307692, -295.4353501694183706, -234.6111521316276196 ) ) ;
#75222=CARTESIAN_POINT ( 'NONE',  ( 26.89796567893247925, -279.7521574817377541, -234.6608544840322566 ) ) ;
#75223=CARTESIAN_POINT ( 'NONE',  ( -10.95739305308923583, -272.4785094481035230, -200.6986525670266133 ) ) ;
#75224=CARTESIAN_POINT ( 'NONE',  ( -20.72046952621861493, -296.1496045391317011, -342.0025305447263690 ) ) ;
#75226=CARTESIAN_POINT ( 'NONE',  ( -23.49674637501712127, -296.7023972115603101, -194.0579500639032062 ) ) ;
#75227=CARTESIAN_POINT ( 'NONE',  ( 35.39309751281768968, -292.0737742304446556, -292.5306180513165941 ) ) ;
#75228=CARTESIAN_POINT ( 'NONE',  ( -22.64051395442955084, -293.6693083814956822, -198.2552926939281690 ) ) ;
#75230=CARTESIAN_POINT ( 'NONE',  ( 35.80382008721097975, -294.3961171214106116, -273.4856931472226051 ) ) ;
#75232=CARTESIAN_POINT ( 'NONE',  ( -37.34015228191829294, -281.0722095964095502, -345.7291079347724008 ) ) ;
#75233=CARTESIAN_POINT ( 'NONE',  ( 30.58556167352163868, -293.9113567539073415, -297.2367953213710052 ) ) ;
#75234=CARTESIAN_POINT ( 'NONE',  ( 31.07714474574143537, -282.0074994817105676, -305.6862034903373342 ) ) ;
#75235=CARTESIAN_POINT ( 'NONE',  ( 32.97520123358409450, -283.1133696276980345, -242.5625521931111166 ) ) ;
#75236=CARTESIAN_POINT ( 'NONE',  ( -18.18318485867174417, -285.9591214211972670, -195.7493696748659886 ) ) ;
#75237=CARTESIAN_POINT ( 'NONE',  ( -102.7131092270129642, -289.0390828449675382, -233.8321282387747715 ) ) ;
#75238=CARTESIAN_POINT ( 'NONE',  ( -33.11666398719405890, -281.4797592383476967, -346.5637458061077041 ) ) ;
#75239=CARTESIAN_POINT ( 'NONE',  ( 37.98914964576849229, -286.2919313450086065, -255.9821200031829846 ) ) ;
#75241=CARTESIAN_POINT ( 'NONE',  ( -34.24747818468571126, -296.6127322976963683, -344.0962263578530838 ) ) ;
#75242=CARTESIAN_POINT ( 'NONE',  ( 36.32245510802563615, -277.2342699753088482, -290.7126212003955175 ) ) ;
#75243=CARTESIAN_POINT ( 'NONE',  ( 37.22807805006183912, -291.4291010117114524, -259.1587148546435628 ) ) ;
#75244=CARTESIAN_POINT ( 'NONE',  ( -87.54208127033960807, -278.9950118524668028, -217.2628624188239428 ) ) ;
#75245=CARTESIAN_POINT ( 'NONE',  ( 30.89793999602319019, -293.2573319643981904, -234.5763028660053919 ) ) ;
#75246=CARTESIAN_POINT ( 'NONE',  ( -112.7134655645136121, -282.7087573052382368, -264.3382097483162738 ) ) ;
#75247=CARTESIAN_POINT ( 'NONE',  ( -15.15634930496033839, -278.7651667279599224, -342.0591375166766852 ) ) ;
#75248=CARTESIAN_POINT ( 'NONE',  ( 18.14287874211904494, -293.2896744372609419, -318.1805482482629372 ) ) ;
#75249=CARTESIAN_POINT ( 'NONE',  ( -9.995406632704115779, -296.3943103766233662, -195.3704328563498223 ) ) ;
#75252=CARTESIAN_POINT ( 'NONE',  ( -68.00448871744069379, -281.6275074730502865, -202.2910477437457075 ) ) ;
#75253=CARTESIAN_POINT ( 'NONE',  ( 34.01126211579226322, -292.8520000139972694, -254.5951841277714323 ) ) ;
#75255=CARTESIAN_POINT ( 'NONE',  ( -110.4542110544635705, -276.2666405000204009, -253.6410175316879361 ) ) ;
#75256=CARTESIAN_POINT ( 'NONE',  ( -68.07221948050482752, -296.7173024705481339, -199.9592402143491654 ) ) ;
#75257=CARTESIAN_POINT ( 'NONE',  ( 9.936434745182769035, -289.7317894805787546, -330.5789735285498523 ) ) ;
#75258=CARTESIAN_POINT ( 'NONE',  ( 12.15424199531149085, -288.1740223768405826, -324.0875322261592828 ) ) ;
#75259=CARTESIAN_POINT ( 'NONE',  ( -71.27802072453108906, -281.1157834562762901, -204.9325702088000014 ) ) ;
#75260=CARTESIAN_POINT ( 'NONE',  ( -96.10712921652623209, -298.9368236130865739, -225.3449228262869042 ) ) ;
#75261=CARTESIAN_POINT ( 'NONE',  ( -69.90270273723888295, -278.4083762322092639, -204.5679346886585677 ) ) ;
#75263=CARTESIAN_POINT ( 'NONE',  ( -26.20926470230388361, -297.8546836819828059, -193.3828706296505686 ) ) ;
#75264=CARTESIAN_POINT ( 'NONE',  ( -52.69009729901044636, -293.7742849741289888, -197.4676726259614270 ) ) ;
#75265=CARTESIAN_POINT ( 'NONE',  ( 25.85972067148311737, -295.7189814082070711, -312.9289558919719525 ) ) ;
#75268=CARTESIAN_POINT ( 'NONE',  ( -101.2167761406611532, -291.6902297003558715, -234.7062159187138377 ) ) ;
#75270=CARTESIAN_POINT ( 'NONE',  ( 38.00051562053408816, -291.5840409800447901, -261.8879754339709507 ) ) ;
#75271=CARTESIAN_POINT ( 'NONE',  ( -99.32937735309978677, -272.5931160627417853, -231.6892119803141270 ) ) ;
#75272=CARTESIAN_POINT ( 'NONE',  ( -97.60007241036942105, -291.4413513588268643, -317.1760336096171500 ) ) ;
#75273=CARTESIAN_POINT ( 'NONE',  ( -19.11405058567862625, -288.7662352645559167, -190.3538533559490702 ) ) ;
#75274=CARTESIAN_POINT ( 'NONE',  ( 35.15855799789352432, -289.3129832592465505, -251.7692137556176704 ) ) ;
#75275=CARTESIAN_POINT ( 'NONE',  ( -3.247226104629870491, -272.5032799758094484, -203.7314525690737241 ) ) ;
#75276=CARTESIAN_POINT ( 'NONE',  ( 35.23229767130369083, -277.2573763744300663, -253.7413302163571984 ) ) ;
#75277=CARTESIAN_POINT ( 'NONE',  ( -41.65224650118132388, -290.0774172856012001, -195.9951922068460135 ) ) ;
#75278=CARTESIAN_POINT ( 'NONE',  ( -108.4551717096112640, -280.7500177086495796, -244.0718165073823513 ) ) ;
#75280=CARTESIAN_POINT ( 'NONE',  ( -32.14672447486484685, -282.3334752730351624, -343.2782277459201623 ) ) ;
#75281=CARTESIAN_POINT ( 'NONE',  ( -113.4123183080833002, -279.7591301606798311, -260.2224168589726219 ) ) ;
#75282=CARTESIAN_POINT ( 'NONE',  ( -3.817452920253944892, -279.2795266825058320, -201.4690018977922534 ) ) ;
#75283=CARTESIAN_POINT ( 'NONE',  ( 172.0454967774839758, 241.8891635430174460, -177.5408160709527294 ) ) ;
#75284=CARTESIAN_POINT ( 'NONE',  ( 23.43917387236569994, -275.8654640167657703, -223.4515018542266489 ) ) ;
#75286=CARTESIAN_POINT ( 'NONE',  ( -65.98508653526388912, -275.2042228488130604, -199.6203872412735620 ) ) ;
#75287=CARTESIAN_POINT ( 'NONE',  ( 27.33386217378599881, -277.6233781216988064, -239.1787733560258573 ) ) ;
#75292=CARTESIAN_POINT ( 'NONE',  ( -104.3245834902642315, -291.2309609334361653, -300.2776941623626499 ) ) ;
#75293=CARTESIAN_POINT ( 'NONE',  ( -86.70884949778225348, -291.4873085994771600, -328.1957597084564782 ) ) ;
#75294=CARTESIAN_POINT ( 'NONE',  ( -110.4085784052586234, -289.8540419052837365, -273.9056393316333811 ) ) ;
#75295=CARTESIAN_POINT ( 'NONE',  ( 14.21030148547296257, -286.2608757155883268, -213.1764317135298654 ) ) ;
#75297=CARTESIAN_POINT ( 'NONE',  ( 24.79310128011774594, -280.4980631039326795, -310.2759600145307672 ) ) ;
#75298=CARTESIAN_POINT ( 'NONE',  ( -29.01138261004551921, -290.8058670193477724, -344.1274469505269735 ) ) ;
#75299=CARTESIAN_POINT ( 'NONE',  ( -96.48969585351893841, -282.4212863938078613, -314.3181692438258210 ) ) ;
#75300=CARTESIAN_POINT ( 'NONE',  ( 34.54407498774808261, -282.6662708677534397, -255.0146650815508451 ) ) ;
#75301=CARTESIAN_POINT ( 'NONE',  ( 36.91984624388441460, -288.7375258160590761, -289.8044444484485780 ) ) ;
#75302=CARTESIAN_POINT ( 'NONE',  ( -74.54251828192542462, -280.0355259030642969, -207.4214289296987488 ) ) ;
#75303=CARTESIAN_POINT ( 'NONE',  ( -101.9745294075216009, -288.8042359777514889, -311.5757410587415279 ) ) ;
#75304=CARTESIAN_POINT ( 'NONE',  ( -110.7747526308671127, -285.6417031317057535, -247.5601590194017376 ) ) ;
#75305=CARTESIAN_POINT ( 'NONE',  ( -54.95661389131981167, -286.3238594502032583, -195.4662468886860722 ) ) ;
#75306=CARTESIAN_POINT ( 'NONE',  ( -97.53114532118206625, -284.1427779865191496, -311.7557601251275514 ) ) ;
#75309=CARTESIAN_POINT ( 'NONE',  ( -42.00203842906732632, -293.8544102891200964, -194.7397801981711609 ) ) ;
#75310=CARTESIAN_POINT ( 'NONE',  ( -16.65641623173852892, -293.4753148378163132, -344.0734252268142654 ) ) ;
#75311=CARTESIAN_POINT ( 'NONE',  ( -35.12247642981180462, -276.0823494035944918, -343.5627811801691678 ) ) ;
#75312=EDGE_CURVE ( 'NONE', #64758, #52349, #43846, .T. ) ;
#75313=CARTESIAN_POINT ( 'NONE',  ( -112.5072827329021123, -295.6974813788014558, -286.5921986236854764 ) ) ;
#75314=CARTESIAN_POINT ( 'NONE',  ( -12.00380657687494157, -290.8677333333762931, -201.1062971438530553 ) ) ;
#75315=CARTESIAN_POINT ( 'NONE',  ( 10.93578421656968835, -292.6131472422081288, -326.4615503911931000 ) ) ;
#75316=CARTESIAN_POINT ( 'NONE',  ( -108.8176499621582849, -291.9768338629787650, -253.6233617919739913 ) ) ;
#75317=CARTESIAN_POINT ( 'NONE',  ( -1.115838972928507866, -293.6246253637290806, -206.6134433889496336 ) ) ;
#75319=CARTESIAN_POINT ( 'NONE',  ( -28.00151579417840964, -292.9338161732316053, -344.9972500138078431 ) ) ;
#75320=CARTESIAN_POINT ( 'NONE',  ( -38.16888550275267278, -297.0626855024811448, -345.3691057194579344 ) ) ;
#75321=CARTESIAN_POINT ( 'NONE',  ( 35.68753111600568673, -288.5739884109801778, -276.4891305649846913 ) ) ;
#75322=CARTESIAN_POINT ( 'NONE',  ( 35.99704987304163240, -277.7539764534426467, -287.7325100432989871 ) ) ;
#75323=CARTESIAN_POINT ( 'NONE',  ( -62.29124493179421052, -276.1643886034883053, -342.8431639951513716 ) ) ;
#75325=CARTESIAN_POINT ( 'NONE',  ( -96.85190254110702313, -272.5556876607107029, -221.6389443325548712 ) ) ;
#75326=CARTESIAN_POINT ( 'NONE',  ( 29.07706990278712311, -279.1831142298798341, -236.6333423517621952 ) ) ;
#75327=CARTESIAN_POINT ( 'NONE',  ( -68.70492063670869243, -275.8574026286449339, -339.8216766797372657 ) ) ;
#75329=CARTESIAN_POINT ( 'NONE',  ( -104.3933690947992403, -294.8329245121622648, -300.5740712314096186 ) ) ;
#75330=CARTESIAN_POINT ( 'NONE',  ( -69.75615881439807708, -275.6256097503289766, -202.7135829966783263 ) ) ;
#75331=CARTESIAN_POINT ( 'NONE',  ( -56.89685064867380504, -274.4447684151328986, -199.8704901249973602 ) ) ;
#75333=CARTESIAN_POINT ( 'NONE',  ( -68.69641587537209659, -287.4823015945534053, -338.8974120948885798 ) ) ;
#75334=CARTESIAN_POINT ( 'NONE',  ( 20.68282252024792101, -274.7622947492533854, -226.0443253088345443 ) ) ;
#75335=CARTESIAN_POINT ( 'NONE',  ( 39.09056570307249245, -287.6742402772570131, -280.1231841771567019 ) ) ;
#75336=CARTESIAN_POINT ( 'NONE',  ( -99.70216693761570070, -275.1197216756281705, -228.3017489483409292 ) ) ;
#75337=CARTESIAN_POINT ( 'NONE',  ( -104.1580704829187027, -294.9995364125176707, -236.5471354320052910 ) ) ;
#75338=CARTESIAN_POINT ( 'NONE',  ( 15.63479333641765834, -281.5222773165192507, -326.0176536307007495 ) ) ;
#75340=CARTESIAN_POINT ( 'NONE',  ( -67.10673074314206588, -277.6619532058171558, -201.4657905397364175 ) ) ;
#75342=CARTESIAN_POINT ( 'NONE',  ( -64.20271485585210769, -290.4886574501826431, -202.0421951684783437 ) ) ;
#75343=CARTESIAN_POINT ( 'NONE',  ( -81.37758304822348521, -281.7973128115350505, -330.1888434668369996 ) ) ;
#75346=CARTESIAN_POINT ( 'NONE',  ( -52.75661796808977044, -289.8546012373262784, -196.9090188413492513 ) ) ;
#75347=CARTESIAN_POINT ( 'NONE',  ( 23.61505529878225929, -276.5014874611289883, -228.9261539381503496 ) ) ;
#75348=CARTESIAN_POINT ( 'NONE',  ( 22.94927417554640314, -283.6095701445305508, -317.3248361464147820 ) ) ;
#75349=CARTESIAN_POINT ( 'NONE',  ( -46.67836583503722636, -272.0143457914076635, -195.3801812718675706 ) ) ;
#75350=CARTESIAN_POINT ( 'NONE',  ( -56.31889993073173883, -283.3035837589264361, -340.8513008994051461 ) ) ;
#75351=CARTESIAN_POINT ( 'NONE',  ( 17.71441209160705910, -276.2845628980930996, -221.4573699871448582 ) ) ;
#75352=CARTESIAN_POINT ( 'NONE',  ( 35.86057388107091981, -276.3710001678674075, -271.5774712844498708 ) ) ;
#75353=CARTESIAN_POINT ( 'NONE',  ( 32.72829147636313962, -283.8999001108152811, -297.1042839005453970 ) ) ;
#75354=CONICAL_SURFACE ( 'NONE', #64864, 2.390969801828402019, 0.09862129276974965220 ) ;
#75357=CARTESIAN_POINT ( 'NONE',  ( 25.71343354142396720, -293.9701106841199589, -314.5774547246325028 ) ) ;
#75358=CARTESIAN_POINT ( 'NONE',  ( -55.17315685265742076, -287.8017243051488094, -197.8239431479683788 ) ) ;
#75360=CARTESIAN_POINT ( 'NONE',  ( -37.30987171927208834, -283.5523547857346784, -190.3611179825600175 ) ) ;
#75361=CARTESIAN_POINT ( 'NONE',  ( -113.9191096521135478, -277.6622799374305259, -277.3062882068961699 ) ) ;
#75362=CARTESIAN_POINT ( 'NONE',  ( -8.791848100974863911, -290.8193944210870541, -199.7116568020229295 ) ) ;
#75363=CARTESIAN_POINT ( 'NONE',  ( -60.21200603465616297, -287.2703344579918507, -200.3064474805385657 ) ) ;
#75365=CARTESIAN_POINT ( 'NONE',  ( -46.00476219779407216, -278.9235134409516945, -343.9170399857970892 ) ) ;
#75366=CARTESIAN_POINT ( 'NONE',  ( -82.93892312404993561, -286.8675972362315747, -208.9803675943674364 ) ) ;
#75367=CARTESIAN_POINT ( 'NONE',  ( 37.12874587794093628, -283.6719962762423393, -279.6821982932442552 ) ) ;
#75368=CARTESIAN_POINT ( 'NONE',  ( 39.31709503734047217, -275.6214960333552426, -262.5782332446160581 ) ) ;
#75369=CARTESIAN_POINT ( 'NONE',  ( -113.2995155449436311, -278.2275700493729573, -282.9868964382306444 ) ) ;
#75371=CARTESIAN_POINT ( 'NONE',  ( -108.0827537339674507, -298.7758212115975311, -247.0238949430231798 ) ) ;
#75373=CARTESIAN_POINT ( 'NONE',  ( 31.98288692825981272, -278.4805209788417528, -303.7098442033569654 ) ) ;
#75374=CARTESIAN_POINT ( 'NONE',  ( -112.0675664805953602, -270.9702663037409707, -256.2959009891208098 ) ) ;
#75376=CARTESIAN_POINT ( 'NONE',  ( -93.65746993446894919, -277.4003203043759527, -316.9266403862098969 ) ) ;
#75377=CARTESIAN_POINT ( 'NONE',  ( 25.80849035868142138, -276.1817352553266574, -226.9781913343555573 ) ) ;
#75378=CARTESIAN_POINT ( 'NONE',  ( 9.057031034392009516, -281.4912993696004833, -331.5164771819336238 ) ) ;
#75379=CARTESIAN_POINT ( 'NONE',  ( 36.66867560463269626, -289.3209148574447340, -271.0231563411240927 ) ) ;
#75380=CARTESIAN_POINT ( 'NONE',  ( -79.08138327671389334, -297.1243357125612761, -334.2399611328908122 ) ) ;
#75381=CARTESIAN_POINT ( 'NONE',  ( -50.38473620873794800, -296.4200609167568246, -345.8991389058134587 ) ) ;
#75382=CARTESIAN_POINT ( 'NONE',  ( -1.585301103958060009, -294.5273562399443108, -204.6083880934220076 ) ) ;
#75383=CARTESIAN_POINT ( 'NONE',  ( -86.67413386912890871, -277.3642737467271218, -214.0908824675673543 ) ) ;
#75384=CARTESIAN_POINT ( 'NONE',  ( -19.20696102403819694, -282.2073331598957111, -198.1105339240040735 ) ) ;
#75385=CARTESIAN_POINT ( 'NONE',  ( -109.2198446831052649, -294.8833523136493113, -250.9511066080622470 ) ) ;
#75386=CARTESIAN_POINT ( 'NONE',  ( -89.87173445043413267, -285.3786451039043754, -325.6334107386399523 ) ) ;
#75387=CARTESIAN_POINT ( 'NONE',  ( 4.914718632275406840, -285.5581694718601966, -210.3938894123811565 ) ) ;
#75388=CARTESIAN_POINT ( 'NONE',  ( -1.176032765980912442, -279.8678231192329235, -202.4983351698289766 ) ) ;
#75389=CARTESIAN_POINT ( 'NONE',  ( -69.20386377067950434, -197.1553935057814329, -359.8476434964631494 ) ) ;
#75391=CARTESIAN_POINT ( 'NONE',  ( -22.45137806013714510, -285.9146668119472565, -198.8223991060767446 ) ) ;
#75393=CARTESIAN_POINT ( 'NONE',  ( -50.02877699809521772, -284.2899392448449021, -346.0489649473844906 ) ) ;
#75394=CARTESIAN_POINT ( 'NONE',  ( 35.60785113091043286, -275.8296825684327018, -266.1335175944963680 ) ) ;
#75395=CARTESIAN_POINT ( 'NONE',  ( 29.79101526281119661, -285.8655537276382006, -233.3564738196167809 ) ) ;
#75396=CARTESIAN_POINT ( 'NONE',  ( -64.26734567658402852, -290.6293759687758325, -198.4963863440569583 ) ) ;
#75397=CARTESIAN_POINT ( 'NONE',  ( 22.68380223392676243, -281.8505438747735639, -222.4887952267571336 ) ) ;
#75399=CARTESIAN_POINT ( 'NONE',  ( -61.84349475687296405, -281.2596210423544676, -198.0394208202278890 ) ) ;
#75400=CARTESIAN_POINT ( 'NONE',  ( 10.80647592606522345, -281.0302018658910015, -210.2303526422367099 ) ) ;
#75401=CARTESIAN_POINT ( 'NONE',  ( -6.941161984400256557, -277.9809262143061233, -207.3071070584150277 ) ) ;
#75402=CARTESIAN_POINT ( 'NONE',  ( -55.52635933303225357, -169.8022349263865465, -364.5488151334876079 ) ) ;
#75403=ORIENTED_EDGE ( 'NONE', *, *, #74502, .F. ) ;
#75404=CARTESIAN_POINT ( 'NONE',  ( 17.90133156924967750, -278.2588308063758404, -320.8602921365193197 ) ) ;
#75405=CARTESIAN_POINT ( 'NONE',  ( 24.53442447440543717, -22.56791868723661310, -344.6573901678291350 ) ) ;
#75406=CARTESIAN_POINT ( 'NONE',  ( 31.54898167787137453, -279.1952580483235806, -241.6222808393749517 ) ) ;
#75407=CARTESIAN_POINT ( 'NONE',  ( -99.97986236466763899, -296.4197585603535003, -232.5751212401761165 ) ) ;
#75408=CARTESIAN_POINT ( 'NONE',  ( -77.13206452982005601, -291.0419367364358436, -204.4494397070376692 ) ) ;
#75410=CARTESIAN_POINT ( 'NONE',  ( -82.60680842947836311, -296.0222551359900081, -208.7350419860082695 ) ) ;
#75411=CARTESIAN_POINT ( 'NONE',  ( 19.28860886320061496, -285.2874478753681160, -223.0186112760830781 ) ) ;
#75412=CARTESIAN_POINT ( 'NONE',  ( 35.54152331504181461, -295.5955191682776899, -284.4643524746339835 ) ) ;
#75413=CARTESIAN_POINT ( 'NONE',  ( -22.37566657928664071, -287.5628567668544520, -198.3557010508719713 ) ) ;
#75415=CARTESIAN_POINT ( 'NONE',  ( 19.23412005513974776, -293.7853309483400039, -218.4766618935138922 ) ) ;
#75416=CARTESIAN_POINT ( 'NONE',  ( -94.32907488382490158, -284.3987133522176691, -316.1022113187067930 ) ) ;
#75417=CARTESIAN_POINT ( 'NONE',  ( -104.8961631381495749, -295.8175168407189517, -234.1321119835277500 ) ) ;
#75418=CARTESIAN_POINT ( 'NONE',  ( -64.34165984888359446, -292.5115763540368903, -198.3664673955713340 ) ) ;
#75419=CARTESIAN_POINT ( 'NONE',  ( -104.5592611150223377, -291.5301760400951139, -232.9268235716128856 ) ) ;
#75420=CARTESIAN_POINT ( 'NONE',  ( -3.364479692689621881, -288.7573924854837060, -335.0278493176429606 ) ) ;
#75423=CARTESIAN_POINT ( 'NONE',  ( -79.95026689803805198, -299.3432684683767775, -207.6496786365150626 ) ) ;
#75424=CARTESIAN_POINT ( 'NONE',  ( -110.6526080846042674, -271.6294500476170697, -247.9646197041413132 ) ) ;
#75425=CARTESIAN_POINT ( 'NONE',  ( 24.32210373110764934, -281.1568332811862660, -309.9636086721840798 ) ) ;
#75427=CARTESIAN_POINT ( 'NONE',  ( -38.55028482043721283, -276.5745819193871284, -347.2900866910381410 ) ) ;
#75429=CARTESIAN_POINT ( 'NONE',  ( -83.67722140541020792, -271.8037732317044970, -212.9201928424127459 ) ) ;
#75430=CARTESIAN_POINT ( 'NONE',  ( -97.07301344490083750, -279.8047577323887367, -314.4622951484155919 ) ) ;
#75431=CARTESIAN_POINT ( 'NONE',  ( -56.94885020070252324, -275.4471545935467134, -342.0135678286415555 ) ) ;
#75432=CARTESIAN_POINT ( 'NONE',  ( -107.9808136697012912, -297.4951821191953059, -290.2921526658607831 ) ) ;
#75433=CARTESIAN_POINT ( 'NONE',  ( -60.62705750101235935, -298.8226808384153514, -200.7946990238000353 ) ) ;
#75434=CARTESIAN_POINT ( 'NONE',  ( -46.05879257339719146, -299.5434698108736598, -194.6613642591835003 ) ) ;
#75435=CARTESIAN_POINT ( 'NONE',  ( -32.75693280770970262, -272.1297432355383421, -195.1326468809630796 ) ) ;
#75436=CARTESIAN_POINT ( 'NONE',  ( 28.48995345694742554, -294.6344645119119718, -302.2597342487869696 ) ) ;
#75437=CARTESIAN_POINT ( 'NONE',  ( 18.93885819975810492, -291.4587117284910391, -222.9493718335389474 ) ) ;
#75439=CARTESIAN_POINT ( 'NONE',  ( 23.58026961463914262, -275.4166318513267129, -223.3498842020389645 ) ) ;
#75440=CARTESIAN_POINT ( 'NONE',  ( -108.5353678881545108, -272.9317305373718341, -254.2222928887280489 ) ) ;
#75441=CARTESIAN_POINT ( 'NONE',  ( -92.09259267088177126, -282.4992613816153266, -323.7992882179617027 ) ) ;
#75443=CARTESIAN_POINT ( 'NONE',  ( -95.25050953846822210, -283.1209787989429856, -315.0936674656495029 ) ) ;
#75444=CARTESIAN_POINT ( 'NONE',  ( -101.3700716200489467, -282.0248365383689588, -309.7361871153909192 ) ) ;
#75446=CARTESIAN_POINT ( 'NONE',  ( -16.22904348933836971, -275.3486658582631890, -340.9101579455689262 ) ) ;
#75447=CARTESIAN_POINT ( 'NONE',  ( 18.82090464115082185, -282.8604287763149046, -220.5785614886872850 ) ) ;
#75450=CARTESIAN_POINT ( 'NONE',  ( -100.5335881872930486, -271.5200136539978644, -227.6852286739031399 ) ) ;
#75451=CARTESIAN_POINT ( 'NONE',  ( -85.89117158931847484, -279.7225441514551676, -327.8136690351561811 ) ) ;
#75453=CARTESIAN_POINT ( 'NONE',  ( -88.92145780250835685, -287.2548237929879633, -215.0736053048038059 ) ) ;
#75455=CARTESIAN_POINT ( 'NONE',  ( -95.85189033846208417, -287.9063580454692328, -317.3019677763954292 ) ) ;
#75456=CARTESIAN_POINT ( 'NONE',  ( -110.4443161140219871, -295.4404229792202159, -263.2459833580459758 ) ) ;
#75457=CARTESIAN_POINT ( 'NONE',  ( -56.40526817440679963, -287.4398563908156348, -342.1602714547207142 ) ) ;
#75458=CARTESIAN_POINT ( 'NONE',  ( -32.04911714649202992, -124.5213432794980974, -365.6788127701597659 ) ) ;
#75459=CARTESIAN_POINT ( 'NONE',  ( -76.22636613857584109, -295.5326814296889779, -206.1683707727777346 ) ) ;
#75460=CARTESIAN_POINT ( 'NONE',  ( 37.61280969453202516, -285.8515519814939694, -256.0597470183237192 ) ) ;
#75461=CARTESIAN_POINT ( 'NONE',  ( 34.84346732286840620, -282.9511790556244932, -254.9470931158175233 ) ) ;
#75462=CARTESIAN_POINT ( 'NONE',  ( -102.0668173571852435, -282.2648171203965717, -310.1685696986380094 ) ) ;
#75463=CARTESIAN_POINT ( 'NONE',  ( -23.78517560321560254, -288.8742271508500608, -342.1430102089080378 ) ) ;
#75464=CARTESIAN_POINT ( 'NONE',  ( 36.29264799876062142, -282.9897620476032216, -271.3033343605562209 ) ) ;
#75465=CARTESIAN_POINT ( 'NONE',  ( 35.68040274552090807, -282.2955766887364462, -265.8473370328452461 ) ) ;
#75466=CARTESIAN_POINT ( 'NONE',  ( 23.36296611403582091, -288.9260064859467434, -225.7141662209383242 ) ) ;
#75467=CARTESIAN_POINT ( 'NONE',  ( -114.3207138216981775, -272.9212413174133189, -267.4986742080367890 ) ) ;
#75469=CARTESIAN_POINT ( 'NONE',  ( -55.33361865955895809, -273.8268481185501173, -195.4926274971984128 ) ) ;
#75470=CARTESIAN_POINT ( 'NONE',  ( 23.92382483820542305, -294.9504984232843867, -227.6961137215915016 ) ) ;
#75472=CARTESIAN_POINT ( 'NONE',  ( -69.85430415644619018, -279.9805209788416391, -337.9475929042657754 ) ) ;
#75474=CARTESIAN_POINT ( 'NONE',  ( 32.47179602852396130, -273.9156722061202345, -298.3599745655197353 ) ) ;
#75476=CARTESIAN_POINT ( 'NONE',  ( -89.05031925654860459, -295.7398368506991346, -214.3194964663088058 ) ) ;
#75477=CARTESIAN_POINT ( 'NONE',  ( -59.49865158884114180, -273.1062489779997691, -200.6449195533147076 ) ) ;
#75478=CARTESIAN_POINT ( 'NONE',  ( -92.92201667035706691, -291.3881049729789652, -318.8267731078408929 ) ) ;
#75479=CARTESIAN_POINT ( 'NONE',  ( -77.39382854392350453, -292.4414631337652963, -209.0485135921806261 ) ) ;
#75480=CARTESIAN_POINT ( 'NONE',  ( 22.64622667818251500, -283.9106732801743078, -313.7351348400027859 ) ) ;
#75481=CARTESIAN_POINT ( 'NONE',  ( -112.7754452456914294, -291.8239159292358522, -282.5412818059990059 ) ) ;
#75482=CARTESIAN_POINT ( 'NONE',  ( -88.33334392329902585, -292.6702770558816837, -213.3247214041538768 ) ) ;
#75483=CARTESIAN_POINT ( 'NONE',  ( 21.32520173268260777, -293.9945727066852328, -313.8029714257997966 ) ) ;
#75484=CARTESIAN_POINT ( 'NONE',  ( 27.43596741592070387, -290.0584838143359434, -308.2640377754182168 ) ) ;
#75485=CARTESIAN_POINT ( 'NONE',  ( 32.39329112684018952, -282.1383118845998865, -303.1368738788993937 ) ) ;
#75486=CARTESIAN_POINT ( 'NONE',  ( -103.9720348149101738, -295.1025535926976318, -234.6171638881198191 ) ) ;
#75487=CARTESIAN_POINT ( 'NONE',  ( -94.40058091006845586, -283.6829267836913573, -322.0844857593970687 ) ) ;
#75488=CARTESIAN_POINT ( 'NONE',  ( 36.24293263423945177, -277.3693427529578912, -257.7494534230675072 ) ) ;
#75490=CARTESIAN_POINT ( 'NONE',  ( -110.6386073502017524, -276.4471613113626063, -289.5920658546791060 ) ) ;
#75492=CARTESIAN_POINT ( 'NONE',  ( 18.53737438131143378, -281.7280861414042761, -317.4498203518813852 ) ) ;
#75493=CARTESIAN_POINT ( 'NONE',  ( -19.86182089997161881, -281.4769613736951328, -195.7247144114786579 ) ) ;
#75494=CARTESIAN_POINT ( 'NONE',  ( 7.416498944221869394, -285.7044324591514055, -207.9295940157504390 ) ) ;
#75495=CARTESIAN_POINT ( 'NONE',  ( 25.69938988429784033, -294.7838866398691948, -231.4850727887573214 ) ) ;
#75496=CARTESIAN_POINT ( 'NONE',  ( 30.52841517487776812, -276.7014170784158296, -235.7188336728002582 ) ) ;
#75498=CARTESIAN_POINT ( 'NONE',  ( 22.36292467856653232, -276.2221205815426401, -222.5004490848821774 ) ) ;
#75499=CARTESIAN_POINT ( 'NONE',  ( -107.8208158827665102, -278.1342603841832783, -289.3793788641613673 ) ) ;
#75501=CARTESIAN_POINT ( 'NONE',  ( -58.44559637772922400, -299.7788533558973540, -198.5651989685439105 ) ) ;
#75502=CARTESIAN_POINT ( 'NONE',  ( 36.94106174778084295, -285.6685888657775649, -279.4220072260627035 ) ) ;
#75503=CARTESIAN_POINT ( 'NONE',  ( -30.59703257196175841, -294.6357889647652541, -347.0439306009369602 ) ) ;
#75504=CARTESIAN_POINT ( 'NONE',  ( -72.78351026826467773, -291.1136839774639498, -337.8317681975417486 ) ) ;
#75505=CARTESIAN_POINT ( 'NONE',  ( 11.14551424664102264, -291.6624211656057923, -215.3095878084267554 ) ) ;
#75507=CARTESIAN_POINT ( 'NONE',  ( 21.82433282734990598, -292.6201021311567843, -227.5441993546482422 ) ) ;
#75509=CARTESIAN_POINT ( 'NONE',  ( -8.337244887857906406, -289.7608717291013249, -341.3699342028843375 ) ) ;
#75510=CARTESIAN_POINT ( 'NONE',  ( -81.35585617356750276, -280.0873078208157949, -211.9310644025564727 ) ) ;
#75511=CARTESIAN_POINT ( 'NONE',  ( -113.8114384287864453, -295.5538293187850059, -263.8828272511983073 ) ) ;
#75512=CARTESIAN_POINT ( 'NONE',  ( 21.41650567535096172, -288.8727355960625118, -319.9674284450643995 ) ) ;
#75513=CARTESIAN_POINT ( 'NONE',  ( 23.84204542667185933, -287.2621871429266207, -223.6244821193059238 ) ) ;
#75514=CARTESIAN_POINT ( 'NONE',  ( -94.29883822965433637, -284.2396730946844627, -316.0753385126189414 ) ) ;
#75515=CARTESIAN_POINT ( 'NONE',  ( 44.85892074982627520, 12.63905672353519272, -331.9659920184308248 ) ) ;
#75516=CARTESIAN_POINT ( 'NONE',  ( 198.0048462530024835, 289.0459362520341529, -97.09714635992116882 ) ) ;
#75517=CARTESIAN_POINT ( 'NONE',  ( -98.40372196300425855, -246.1885688021466763, -331.2951966265923147 ) ) ;
#75518=CARTESIAN_POINT ( 'NONE',  ( -37.82105694835537690, -276.2554370994141095, -343.5335049148077360 ) ) ;
#75519=CARTESIAN_POINT ( 'NONE',  ( 35.68744478371312567, -274.3810996434528420, -263.4050330088518876 ) ) ;
#75520=CARTESIAN_POINT ( 'NONE',  ( -112.4217224872212881, -272.4314421411885405, -253.3689275932013345 ) ) ;
#75521=CARTESIAN_POINT ( 'NONE',  ( 162.0739375835457281, 217.5763800931431149, -202.8919388766017278 ) ) ;
#75522=CARTESIAN_POINT ( 'NONE',  ( -2.961819958517478923, -275.2922904668048432, -338.7227716373371891 ) ) ;
#75523=CARTESIAN_POINT ( 'NONE',  ( -34.01728514677294157, -275.8546823244878397, -196.4224793688113664 ) ) ;
#75524=VERTEX_POINT ( 'NONE', #90856 ) ;
#75525=CARTESIAN_POINT ( 'NONE',  ( -107.0088747935059956, -290.7509747666633757, -292.5391565758814068 ) ) ;
#75526=CARTESIAN_POINT ( 'NONE',  ( -36.19766262801284995, -298.8689617876239595, -193.5224416173093402 ) ) ;
#75527=CARTESIAN_POINT ( 'NONE',  ( -107.1079312135632193, -296.6290083186109428, -302.7987489562058272 ) ) ;
#75528=CARTESIAN_POINT ( 'NONE',  ( 14.31777978567131271, -294.4679853012818285, -322.0102727936088627 ) ) ;
#75530=CARTESIAN_POINT ( 'NONE',  ( -3.350576749848003910, -278.5270951069018679, -337.8582451197406726 ) ) ;
#75531=CARTESIAN_POINT ( 'NONE',  ( -5.486724394857766640, -282.1518654395823660, -340.3953055234222234 ) ) ;
#75533=CARTESIAN_POINT ( 'NONE',  ( -109.9298667100904510, -279.7711835162901934, -259.7524929787789461 ) ) ;
#75534=CARTESIAN_POINT ( 'NONE',  ( -51.10676383128398470, -278.9859116570374340, -345.0906103715138329 ) ) ;
#75535=CARTESIAN_POINT ( 'NONE',  ( -52.74081829727114012, -296.4258192511982770, -198.3488129022006490 ) ) ;
#75537=CARTESIAN_POINT ( 'NONE',  ( -90.96640795698880311, -278.0067604918602342, -319.9663575602717174 ) ) ;
#75538=CARTESIAN_POINT ( 'NONE',  ( -81.16669618310218937, -274.2763950910264725, -207.1814360051211565 ) ) ;
#75539=CARTESIAN_POINT ( 'NONE',  ( -26.23281384118568482, -287.5983874803950471, -346.0571609255298995 ) ) ;
#75540=CARTESIAN_POINT ( 'NONE',  ( 14.62250010335176320, -276.7838768361430084, -216.2804140178161276 ) ) ;
#75541=CARTESIAN_POINT ( 'NONE',  ( 37.32598281151900466, -274.3321727037697428, -286.6500436654783357 ) ) ;
#75543=CARTESIAN_POINT ( 'NONE',  ( -66.40255638834896956, -288.6397127836306140, -337.5574081931004002 ) ) ;
#75544=CARTESIAN_POINT ( 'NONE',  ( -114.2243790779740493, -283.9414484010326873, -267.1104305919835724 ) ) ;
#75545=CARTESIAN_POINT ( 'NONE',  ( -6.856294350873071153, -280.8863254607354634, -337.8184333113400726 ) ) ;
#75546=CARTESIAN_POINT ( 'NONE',  ( 35.61943195404269602, -279.9963577087116846, -260.3873852803664590 ) ) ;
#75547=CARTESIAN_POINT ( 'NONE',  ( -110.3362999244276921, -282.8208447903838305, -255.7630838256315542 ) ) ;
#75549=CARTESIAN_POINT ( 'NONE',  ( -102.1093901187677631, -292.0459073519975846, -308.2800806593347716 ) ) ;
#75550=CARTESIAN_POINT ( 'NONE',  ( -97.20068485962379157, -279.1670777993381876, -312.8568427931883775 ) ) ;
#75552=CARTESIAN_POINT ( 'NONE',  ( 37.63472146234818894, -280.1248233117642599, -284.0340992244089762 ) ) ;
#75553=CARTESIAN_POINT ( 'NONE',  ( 0.7755028547181611609, -296.5439030358364789, -334.9527543265875806 ) ) ;
#75554=CARTESIAN_POINT ( 'NONE',  ( -68.23968056714322472, -277.8917835280247459, -200.9258260093619413 ) ) ;
#75555=CIRCLE ( 'NONE', #19596, 2.336627660646517501 ) ;
#75556=CARTESIAN_POINT ( 'NONE',  ( -95.34884929620213256, -278.5785463339040575, -314.8477824328130055 ) ) ;
#75557=CARTESIAN_POINT ( 'NONE',  ( -35.90799773116832228, -285.0343997545045909, -345.5269191039802763 ) ) ;
#75559=CARTESIAN_POINT ( 'NONE',  ( -110.1477862413914011, -292.2142253722082046, -290.5746783988967081 ) ) ;
#75560=CARTESIAN_POINT ( 'NONE',  ( 21.97205936250373171, -286.0916722070055016, -221.5140427754677717 ) ) ;
#75561=CARTESIAN_POINT ( 'NONE',  ( -64.34556793961483834, -290.0936685552413792, -201.6653334189272471 ) ) ;
#75563=CARTESIAN_POINT ( 'NONE',  ( 9.968811875681153012, -275.0689077901557198, -326.6013076209559927 ) ) ;
#75564=CARTESIAN_POINT ( 'NONE',  ( -45.24540603004871286, -293.2927583535905001, -344.2257062649113095 ) ) ;
#75567=CARTESIAN_POINT ( 'NONE',  ( 21.68535148986741845, -291.3767933418693019, -222.0029239246068187 ) ) ;
#75568=CARTESIAN_POINT ( 'NONE',  ( -106.3198232020318130, -286.4988033804119709, -244.1226166710571874 ) ) ;
#75569=CARTESIAN_POINT ( 'NONE',  ( -31.92173493456361300, -287.2246484879873947, -346.2061088682024774 ) ) ;
#75570=CARTESIAN_POINT ( 'NONE',  ( -35.94030054764591853, -287.4953448964360518, -196.7852320008686036 ) ) ;
#75572=CARTESIAN_POINT ( 'NONE',  ( 16.13596863575206442, -289.0721462814268534, -320.3626107389182494 ) ) ;
#75573=CARTESIAN_POINT ( 'NONE',  ( 22.65013893752675145, -294.9108322113206668, -224.7396072971405090 ) ) ;
#75575=CARTESIAN_POINT ( 'NONE',  ( 9.555495966421391429, -287.8862709523839953, -209.7916395636346749 ) ) ;
#75576=CARTESIAN_POINT ( 'NONE',  ( -77.07880479656978423, -275.6596411057477667, -334.6891594915077803 ) ) ;
#75577=CARTESIAN_POINT ( 'NONE',  ( -97.90964294489629083, -278.2501198563418257, -317.8718388211117940 ) ) ;
#75578=CARTESIAN_POINT ( 'NONE',  ( -5.194173601533837115, -290.5518041158099436, -201.9809253793999062 ) ) ;
#75579=CARTESIAN_POINT ( 'NONE',  ( -56.55665423666910385, -279.8112414680044822, -195.7421482812434874 ) ) ;
#75580=CARTESIAN_POINT ( 'NONE',  ( -104.0125327661936439, -298.9789486562990533, -236.6774143496517411 ) ) ;
#75582=CARTESIAN_POINT ( 'NONE',  ( -110.3054443252012362, -282.7755235712349418, -252.9481042794747907 ) ) ;
#75583=CARTESIAN_POINT ( 'NONE',  ( -110.3882400659495033, -273.0210997072354075, -270.3670888080694112 ) ) ;
#75584=CARTESIAN_POINT ( 'NONE',  ( -110.8413992618360737, -276.8315705250254268, -259.5812321447068598 ) ) ;
#75585=CARTESIAN_POINT ( 'NONE',  ( 34.55395801893807572, -279.8291311987075574, -291.8940776148406826 ) ) ;
#75586=CARTESIAN_POINT ( 'NONE',  ( -42.77628441597607889, -275.5994431365209039, -346.4740146987608114 ) ) ;
#75587=CARTESIAN_POINT ( 'NONE',  ( -72.43788831395643513, -297.0456299846624688, -335.1749445751922281 ) ) ;
#75588=CARTESIAN_POINT ( 'NONE',  ( -5.596071932459578235, -281.5646362357951489, -340.1730625288862484 ) ) ;
#75589=CARTESIAN_POINT ( 'NONE',  ( -110.6193688495461345, -297.4787155192013302, -271.4786303251781874 ) ) ;
#75590=CARTESIAN_POINT ( 'NONE',  ( -51.72443379259166818, -299.1871589961564837, -195.1643586863121982 ) ) ;
#75591=CARTESIAN_POINT ( 'NONE',  ( -59.47801267278511261, -273.4243297800937285, -200.7231899841992515 ) ) ;
#75592=CARTESIAN_POINT ( 'NONE',  ( 18.20267363971293761, -294.8486975109893820, -219.8883203971818148 ) ) ;
#75593=CARTESIAN_POINT ( 'NONE',  ( 39.64000551281363016, -287.6978412453868827, -268.6827255662338985 ) ) ;
#75594=CARTESIAN_POINT ( 'NONE',  ( -110.9925362049629598, -276.8471102391508794, -253.4830686850930022 ) ) ;
#75595=CARTESIAN_POINT ( 'NONE',  ( -90.78440842374472197, -291.1528845215802903, -214.8535836960148515 ) ) ;
#75596=CARTESIAN_POINT ( 'NONE',  ( 16.17473577180080824, -287.3283430989260410, -320.4293012437802872 ) ) ;
#75597=CARTESIAN_POINT ( 'NONE',  ( -44.67545329771427731, -289.9593064398290494, -195.6689869793197829 ) ) ;
#75599=CARTESIAN_POINT ( 'NONE',  ( 197.0349383350915105, 285.8449894349855640, -111.9383547020201064 ) ) ;
#75600=CARTESIAN_POINT ( 'NONE',  ( -68.79014287673274453, -288.9847860389822358, -336.3079442182998378 ) ) ;
#75602=CARTESIAN_POINT ( 'NONE',  ( -114.1191699866896130, -285.4621353624736457, -272.8535896670638294 ) ) ;
#75603=CARTESIAN_POINT ( 'NONE',  ( 33.11320743190675842, -292.2213349698519664, -239.8828271342735263 ) ) ;
#75604=CARTESIAN_POINT ( 'NONE',  ( -4.025973531531053418, -282.0842764504088223, -201.8157177411264342 ) ) ;
#75606=CARTESIAN_POINT ( 'NONE',  ( -2.628955654622771476, -281.8166113933995689, -202.1678702321460150 ) ) ;
#75607=CARTESIAN_POINT ( 'NONE',  ( -86.93039352514583129, -283.5985774135995143, -324.0022979817832720 ) ) ;
#75608=CARTESIAN_POINT ( 'NONE',  ( -109.4375384162540428, -296.2084115790212309, -297.5520761096885849 ) ) ;
#75609=CARTESIAN_POINT ( 'NONE',  ( -87.68321915755521445, -274.6467622389861276, -216.7472846845810466 ) ) ;
#75610=CARTESIAN_POINT ( 'NONE',  ( 35.56157207631360251, -291.3646958269602578, -254.2719629792056253 ) ) ;
#75611=CARTESIAN_POINT ( 'NONE',  ( -60.60099853117307589, -296.6636858989128314, -200.7859825983607038 ) ) ;
#75614=CARTESIAN_POINT ( 'NONE',  ( -94.37381194975721144, -287.1384832664475084, -222.5212557131695235 ) ) ;
#75615=CARTESIAN_POINT ( 'NONE',  ( 22.93727962674821796, -295.2686063970570558, -317.7946071113971698 ) ) ;
#75616=CARTESIAN_POINT ( 'NONE',  ( -101.0842615080306501, -285.6937978764972854, -234.4693920906954929 ) ) ;
#75617=CARTESIAN_POINT ( 'NONE',  ( 37.67317811608269551, -274.8161146696110109, -286.7193684492440866 ) ) ;
#75618=CARTESIAN_POINT ( 'NONE',  ( 27.96140394629875914, -293.6705370729663400, -229.6548877418164807 ) ) ;
#75619=CARTESIAN_POINT ( 'NONE',  ( -4.011029042539628442, -284.6265726013100448, -202.3073330086760393 ) ) ;
#75621=CARTESIAN_POINT ( 'NONE',  ( -11.16443524875701954, -292.7173091475025899, -197.9138331013843413 ) ) ;
#75622=CARTESIAN_POINT ( 'NONE',  ( -71.17878848368118838, -289.8449971651592705, -335.0833499140610456 ) ) ;
#75625=CARTESIAN_POINT ( 'NONE',  ( -105.1350182532626718, -260.3806308838838959, -315.5284000272559410 ) ) ;
#75626=CARTESIAN_POINT ( 'NONE',  ( -102.3174723830525750, -285.5445516917910709, -310.3718261940808816 ) ) ;
#75627=CARTESIAN_POINT ( 'NONE',  ( -115.3430155898818299, -275.8380690714489560, -288.1317622949166548 ) ) ;
#75629=CARTESIAN_POINT ( 'NONE',  ( -91.90427036224906487, -282.7745485682152093, -319.3407302205261544 ) ) ;
#75630=CARTESIAN_POINT ( 'NONE',  ( -111.7095002220548707, -278.4684188084473249, -250.4312396981229085 ) ) ;
#75631=CARTESIAN_POINT ( 'NONE',  ( -71.80817234150255501, -281.5957443637915389, -203.9231040330332689 ) ) ;
#75632=CARTESIAN_POINT ( 'NONE',  ( 162.8546122839350403, 218.1056854647095236, -203.8705316301375774 ) ) ;
#75633=CARTESIAN_POINT ( 'NONE',  ( 21.14719141989809614, -280.7940828509410949, -319.5307820050714440 ) ) ;
#75634=CARTESIAN_POINT ( 'NONE',  ( 33.40741838781508477, -285.2630762879289819, -246.5617685939234889 ) ) ;
#75635=CARTESIAN_POINT ( 'NONE',  ( -51.63231078431872589, -299.6320545980326528, -195.6767165542249245 ) ) ;
#75636=CARTESIAN_POINT ( 'NONE',  ( -86.52678036557627195, -296.2502273313650107, -324.3871887590011056 ) ) ;
#75638=CARTESIAN_POINT ( 'NONE',  ( 34.13126325227502633, -292.0120806445708013, -253.1941790877583287 ) ) ;
#75639=CARTESIAN_POINT ( 'NONE',  ( -22.94983159419836127, -277.5242185744853600, -345.9545391471402809 ) ) ;
#75640=CARTESIAN_POINT ( 'NONE',  ( -48.87543607973791637, -273.9012764497288686, -198.2268470693725533 ) ) ;
#75641=CARTESIAN_POINT ( 'NONE',  ( 25.89749349388204891, -273.8973568763689741, -226.9523902113789688 ) ) ;
#75643=CARTESIAN_POINT ( 'NONE',  ( -60.77366303512233259, -271.7480946324538991, -199.0618446551372074 ) ) ;
#75644=CARTESIAN_POINT ( 'NONE',  ( -61.38878195573088448, -296.7836181382269842, -342.9446551372978433 ) ) ;
#75647=CARTESIAN_POINT ( 'NONE',  ( -105.4962559509446578, -285.2704820234149565, -297.5026165127687818 ) ) ;
#75648=CARTESIAN_POINT ( 'NONE',  ( 37.87148765206244150, -283.4493427249642536, -281.1754786946539753 ) ) ;
#75649=CARTESIAN_POINT ( 'NONE',  ( -110.4109664734769325, -283.9295207002436428, -268.1759443989990359 ) ) ;
#75650=CARTESIAN_POINT ( 'NONE',  ( -18.83580362120691021, -275.2097468847273376, -341.8032078706576158 ) ) ;
#75651=CARTESIAN_POINT ( 'NONE',  ( -1.817076402661904622, -284.4367422749386378, -335.5589818411642682 ) ) ;
#75652=CARTESIAN_POINT ( 'NONE',  ( -76.74272308500547979, -276.0695467329869075, -332.6968766596721139 ) ) ;
#75653=CARTESIAN_POINT ( 'NONE',  ( 0.7614402486004525628, -275.6530691849285404, -207.7322367299512393 ) ) ;
#75655=CARTESIAN_POINT ( 'NONE',  ( -108.3672986922079531, -279.7283784804499192, -241.0434924193680502 ) ) ;
#75657=DIRECTION ( 'NONE',  ( -1.000000000000000000, -0.000000000000000000, -0.000000000000000000 ) ) ;
#75658=CARTESIAN_POINT ( 'NONE',  ( -111.9168309691474690, -286.2389262482744243, -284.0223615257261258 ) ) ;
#75659=CARTESIAN_POINT ( 'NONE',  ( 17.19412622853532824, -293.4456276253310421, -319.1493105483372688 ) ) ;
#75660=CARTESIAN_POINT ( 'NONE',  ( -104.5168979631347526, -290.3865997928229490, -232.9337806188935076 ) ) ;
#75661=CARTESIAN_POINT ( 'NONE',  ( 31.41839514244654907, -286.1550643673737113, -297.8857912562353931 ) ) ;
#75662=CARTESIAN_POINT ( 'NONE',  ( 35.15101999619818685, -285.9574891468421356, -257.4170380447608295 ) ) ;
#75663=CARTESIAN_POINT ( 'NONE',  ( -110.7014682631587306, -288.9246336265083528, -260.1676451368796847 ) ) ;
#75664=CARTESIAN_POINT ( 'NONE',  ( -83.02996685808358279, -284.8983164834764921, -327.8694507334673744 ) ) ;
#75665=CARTESIAN_POINT ( 'NONE',  ( 37.63225285613200555, -273.5266078951023587, -268.3844997456997703 ) ) ;
#75666=CARTESIAN_POINT ( 'NONE',  ( 38.54884860006462333, -286.0387249353732386, -277.2215135863347655 ) ) ;
#75667=CARTESIAN_POINT ( 'NONE',  ( 30.88186307268721364, -289.1419799849931564, -239.0826013017536411 ) ) ;
#75668=CARTESIAN_POINT ( 'NONE',  ( 34.62262094288523429, -285.8316026612118321, -292.1121043758279257 ) ) ;
#75669=CARTESIAN_POINT ( 'NONE',  ( -61.60139569022783235, -284.3163507508396606, -339.5149967977421852 ) ) ;
#75670=CARTESIAN_POINT ( 'NONE',  ( -12.79770663512714712, -290.7341651381075849, -341.4622770843610624 ) ) ;
#75673=CARTESIAN_POINT ( 'NONE',  ( -100.3624193321353602, -299.0313208375330873, -228.6517799104587709 ) ) ;
#75674=CARTESIAN_POINT ( 'NONE',  ( -2.189757884915854547, -278.5172269357741470, -204.0944431433552211 ) ) ;
#75675=CARTESIAN_POINT ( 'NONE',  ( 22.09087532058367742, -292.0939666494101630, -221.6586765984672809 ) ) ;
#75676=CARTESIAN_POINT ( 'NONE',  ( -72.02312609100363261, -295.9854514089758482, -205.2035463487816003 ) ) ;
#75677=CARTESIAN_POINT ( 'NONE',  ( 35.84508245194749776, -280.1420811450055908, -263.1192938982639475 ) ) ;
#75678=CARTESIAN_POINT ( 'NONE',  ( -4.654090668539102360, -272.5659843010729446, -203.4677660792073368 ) ) ;
#75679=CARTESIAN_POINT ( 'NONE',  ( -66.23167315409401112, -296.7536390291173802, -337.9378368839156224 ) ) ;
#75681=CARTESIAN_POINT ( 'NONE',  ( -48.84617149401242386, -296.3881850962467297, -194.8734951278480878 ) ) ;
#75682=CARTESIAN_POINT ( 'NONE',  ( -11.42418782859369664, -292.9590987485843812, -341.8470178889565432 ) ) ;
#75683=CARTESIAN_POINT ( 'NONE',  ( 18.91540504087728181, -294.3087952890889483, -222.9215455076601415 ) ) ;
#75685=CARTESIAN_POINT ( 'NONE',  ( -14.80635326471109359, -293.1545935799424569, -200.7568087163612915 ) ) ;
#75688=CARTESIAN_POINT ( 'NONE',  ( -78.28759442156885484, -281.6201749803213943, -333.6212202725016596 ) ) ;
#75689=CARTESIAN_POINT ( 'NONE',  ( -80.15477576422820505, -295.6502543090251152, -329.4884429226718225 ) ) ;
#75690=CARTESIAN_POINT ( 'NONE',  ( -1.634139488952519592, -282.5921031205814984, -338.5811305390154757 ) ) ;
#75692=CARTESIAN_POINT ( 'NONE',  ( -29.46088157494614990, -285.8161137574834925, -193.7867293762930387 ) ) ;
#75693=CARTESIAN_POINT ( 'NONE',  ( -110.4593650553174626, -288.3462594590014874, -286.3529994562124443 ) ) ;
#75695=CARTESIAN_POINT ( 'NONE',  ( 17.31601092809237841, -280.7694483825137013, -323.6835921970004506 ) ) ;
#75696=CARTESIAN_POINT ( 'NONE',  ( 31.40421023157099967, -286.9124344535072737, -304.4733753652319024 ) ) ;
#75698=CARTESIAN_POINT ( 'NONE',  ( 20.33158342059506296, -295.7958307762324921, -316.4272565429639599 ) ) ;
#75699=CARTESIAN_POINT ( 'NONE',  ( -45.56800190211330204, -278.5795949427916867, -346.3804354287603360 ) ) ;
#75700=CARTESIAN_POINT ( 'NONE',  ( -94.80486466489504949, -278.8541698223959884, -225.2846716162187874 ) ) ;
#75702=CARTESIAN_POINT ( 'NONE',  ( -30.69938480181331641, -292.3004721418380996, -193.5953904363667277 ) ) ;
#75703=CARTESIAN_POINT ( 'NONE',  ( -109.3213795032796583, -282.3370553878491478, -293.3873016353512071 ) ) ;
#75704=CARTESIAN_POINT ( 'NONE',  ( -101.8716609544143097, -280.0399051702174802, -308.6844275771397292 ) ) ;
#75706=CARTESIAN_POINT ( 'NONE',  ( -3.516960721587788719, -291.5689516074891685, -205.4050139368606267 ) ) ;
#75707=CARTESIAN_POINT ( 'NONE',  ( -111.7864220875513155, -294.6689553751812696, -261.2515614402256006 ) ) ;
#75710=CARTESIAN_POINT ( 'NONE',  ( 22.98025734727558245, -293.6339754671553237, -311.6715371890010147 ) ) ;
#75712=CARTESIAN_POINT ( 'NONE',  ( 17.40634833298269157, -284.4094976428775112, -226.7417163044926838 ) ) ;
#75713=CARTESIAN_POINT ( 'NONE',  ( -29.07902934490101288, -297.2119807634421704, -193.5976933739872266 ) ) ;
#75714=CARTESIAN_POINT ( 'NONE',  ( -67.01335932154566422, -286.9864365401885493, -199.8423905823315749 ) ) ;
#75715=CARTESIAN_POINT ( 'NONE',  ( -3.368263168884978676, -288.4240865118439388, -335.0298367176197871 ) ) ;
#75716=CARTESIAN_POINT ( 'NONE',  ( -68.31133957715724137, -278.9866277862275297, -337.2449364066092130 ) ) ;
#75717=CARTESIAN_POINT ( 'NONE',  ( -103.9356322629459868, -274.5777690077635498, -238.5540650569657259 ) ) ;
#75718=CARTESIAN_POINT ( 'NONE',  ( -110.7477913952213981, -277.3796275827028239, -267.8796118560917989 ) ) ;
#75720=CARTESIAN_POINT ( 'NONE',  ( -111.8177335754042190, -272.6325626290558830, -250.6040595744685220 ) ) ;
#75721=CARTESIAN_POINT ( 'NONE',  ( -96.07186635792241702, -291.8400784423621985, -316.1209830334568096 ) ) ;
#75722=CARTESIAN_POINT ( 'NONE',  ( 20.68783691572517469, -294.4792001358006246, -220.9548238103238589 ) ) ;
#75725=CARTESIAN_POINT ( 'NONE',  ( -80.46095081314754793, -290.3051638082676504, -329.4547972157160984 ) ) ;
#75727=CARTESIAN_POINT ( 'NONE',  ( 23.00598319888725030, -291.0711452265879302, -224.5307811190980942 ) ) ;
#75728=CARTESIAN_POINT ( 'NONE',  ( -30.49118043164711622, -298.4690047432176243, -193.3818862655401176 ) ) ;
#75729=CARTESIAN_POINT ( 'NONE',  ( -34.47463164901564880, -297.7557351676047119, -197.3401415332614306 ) ) ;
#75732=CARTESIAN_POINT ( 'NONE',  ( -91.09624402796100640, -291.3187812030578243, -324.5940544420357128 ) ) ;
#75733=CARTESIAN_POINT ( 'NONE',  ( 44.71564893372296723, -290.0519495502701943, -270.3284710469131937 ) ) ;
#75734=CARTESIAN_POINT ( 'NONE',  ( -80.38408174780046522, -287.4680793534180907, -209.0816246668871088 ) ) ;
#75735=CARTESIAN_POINT ( 'NONE',  ( -38.07540656457012318, -272.0427788424437949, -195.5313771995554362 ) ) ;
#75736=CARTESIAN_POINT ( 'NONE',  ( 30.47603271662454461, -277.8779679084992154, -301.0542655364614575 ) ) ;
#75737=CARTESIAN_POINT ( 'NONE',  ( -69.62032026370162896, -289.7038170951251459, -203.2694408428101269 ) ) ;
#75738=CARTESIAN_POINT ( 'NONE',  ( -42.69486696654973912, -278.9794353856195812, -345.9365709135371389 ) ) ;
#75741=CARTESIAN_POINT ( 'NONE',  ( 7.850475887748682879, -281.7648971298428364, -327.8849627059589693 ) ) ;
#75742=CARTESIAN_POINT ( 'NONE',  ( -108.2321823212805469, -280.0051727290456256, -241.1030927006030140 ) ) ;
#75743=CARTESIAN_POINT ( 'NONE',  ( 10.58658974830555799, -279.4920924973067713, -210.5362127420374350 ) ) ;
#75744=CARTESIAN_POINT ( 'NONE',  ( 43.64731658108150469, 12.32667446486203389, -329.2959963054772174 ) ) ;
#75745=CARTESIAN_POINT ( 'NONE',  ( 37.40305196647869224, -276.2732887545182052, -252.8099132522576440 ) ) ;
#75747=CARTESIAN_POINT ( 'NONE',  ( -31.33413024532110569, -275.6468135919130873, -194.2781405821475573 ) ) ;
#75748=CARTESIAN_POINT ( 'NONE',  ( 35.78497577281001440, -296.2662352645559167, -287.0191576251351080 ) ) ;
#75754=CARTESIAN_POINT ( 'NONE',  ( -97.59516461942406806, -291.0521959831235677, -312.1413524450476871 ) ) ;
#75755=CARTESIAN_POINT ( 'NONE',  ( 36.72677589446506374, -289.0966188602227476, -253.3377499361083096 ) ) ;
#75756=CARTESIAN_POINT ( 'NONE',  ( -88.73862094798492706, -289.1459851605791300, -322.3442806248777970 ) ) ;
#75757=CARTESIAN_POINT ( 'NONE',  ( -12.71746630148235901, -285.8715566567333326, -197.4695957623152935 ) ) ;
#75759=CARTESIAN_POINT ( 'NONE',  ( 36.15100354033334895, -279.8571726824498000, -263.0925968060599303 ) ) ;
#75760=CARTESIAN_POINT ( 'NONE',  ( 25.29303056442937958, -289.9543190067377623, -310.2077739355467543 ) ) ;
#75761=CARTESIAN_POINT ( 'NONE',  ( -0.9260744269094322023, -281.0391104580084516, -334.4283479660504099 ) ) ;
#75762=CARTESIAN_POINT ( 'NONE',  ( -43.81107896392224177, -281.2840033397203570, -197.1026857099741960 ) ) ;
#75764=CARTESIAN_POINT ( 'NONE',  ( 12.27290671139417277, -289.3220892131961364, -328.9376576589830847 ) ) ;
#75765=CARTESIAN_POINT ( 'NONE',  ( -67.33728138209211522, -280.1402030517718913, -203.7272808318804778 ) ) ;
#75766=CARTESIAN_POINT ( 'NONE',  ( -104.2556355560847976, -289.8330264165567201, -233.0712539019202154 ) ) ;
#75767=CARTESIAN_POINT ( 'NONE',  ( -89.78352293075727175, -286.1376822277202905, -214.1281323630736324 ) ) ;
#75768=CARTESIAN_POINT ( 'NONE',  ( -23.80290198384606271, -286.7128994303685658, -194.5690561745006448 ) ) ;
#75769=CARTESIAN_POINT ( 'NONE',  ( -42.93079811054101924, -283.2911959243219258, -343.1969311162948202 ) ) ;
#75772=CARTESIAN_POINT ( 'NONE',  ( 10.32302065142151370, -294.5618394109116025, -211.4006844012274655 ) ) ;
#75773=CARTESIAN_POINT ( 'NONE',  ( 39.11345194492690069, -292.2723757330883814, -273.1732333752716499 ) ) ;
#75774=CARTESIAN_POINT ( 'NONE',  ( -27.24592100949325513, -273.2422152010747709, -197.7739693503697254 ) ) ;
#75775=CARTESIAN_POINT ( 'NONE',  ( -90.64740119244436301, -295.1321861965166704, -325.8583941265673616 ) ) ;
#75776=CARTESIAN_POINT ( 'NONE',  ( -84.25567128901064962, -289.8728945075252454, -213.5299024365953073 ) ) ;
#75777=CARTESIAN_POINT ( 'NONE',  ( -28.80099573426833359, -293.1823856232198295, -343.9317502568304121 ) ) ;
#75778=CARTESIAN_POINT ( 'NONE',  ( -19.99311056139763565, -293.4850652424813688, -198.9912691879978865 ) ) ;
#75780=CARTESIAN_POINT ( 'NONE',  ( 36.99949668997525976, -291.6943164936869834, -281.4703430961965864 ) ) ;
#75781=CARTESIAN_POINT ( 'NONE',  ( -93.27285309890446285, -297.8560243752332894, -320.4036446848157880 ) ) ;
#75782=CARTESIAN_POINT ( 'NONE',  ( 35.86575157290489813, -288.5380873212598658, -273.7588309075588882 ) ) ;
#75783=CARTESIAN_POINT ( 'NONE',  ( -67.03673063214209549, -279.4193505957185835, -339.6186949564010433 ) ) ;
#75784=CARTESIAN_POINT ( 'NONE',  ( -73.92081615026943098, -276.3218025514231044, -337.6811477355925604 ) ) ;
#75785=CARTESIAN_POINT ( 'NONE',  ( -82.86666355484838675, -296.6445946763698203, -208.3948012186001790 ) ) ;
#75786=CARTESIAN_POINT ( 'NONE',  ( -3.422769643851260035, -274.8377665466923645, -336.1447038572201791 ) ) ;
#75787=CARTESIAN_POINT ( 'NONE',  ( -99.17639361337023729, -277.1976287871859199, -228.8234626275265668 ) ) ;
#75788=CARTESIAN_POINT ( 'NONE',  ( -48.39825944296693194, -275.5903687602177570, -345.8080408774952161 ) ) ;
#75790=CARTESIAN_POINT ( 'NONE',  ( -96.36858252565410510, -273.8075911203138730, -227.1525361581299478 ) ) ;
#75792=CARTESIAN_POINT ( 'NONE',  ( -41.69136755116043247, -287.1267744003523603, -345.6036209785452229 ) ) ;
#75793=CARTESIAN_POINT ( 'NONE',  ( 29.08692807571887329, -274.9758998337271692, -239.9694148806571548 ) ) ;
#75794=CARTESIAN_POINT ( 'NONE',  ( 37.71963002168703127, -287.3367626469164975, -253.1329553641232337 ) ) ;
#75795=CARTESIAN_POINT ( 'NONE',  ( -103.9953226774428856, -275.0127505325787070, -235.5019950587779078 ) ) ;
#75796=CARTESIAN_POINT ( 'NONE',  ( -111.1758283853003633, -294.3951485875724643, -282.5492241632111927 ) ) ;
#75797=CARTESIAN_POINT ( 'NONE',  ( 8.458505545426366012, -279.8583330375108744, -208.5981323667115532 ) ) ;
#75799=CARTESIAN_POINT ( 'NONE',  ( 16.98403680409870731, -278.8256595112727609, -218.5790221729846223 ) ) ;
#75801=CARTESIAN_POINT ( 'NONE',  ( -103.9100376976680167, -289.7621435623385651, -239.4453139845581120 ) ) ;
#75804=CARTESIAN_POINT ( 'NONE',  ( -60.86267007755495939, -289.7468991524940520, -199.0903094513208771 ) ) ;
#75805=CARTESIAN_POINT ( 'NONE',  ( -38.10881773538898187, -275.5624914613856049, -196.6717748918384814 ) ) ;
#75806=CARTESIAN_POINT ( 'NONE',  ( -16.28664212961364655, -284.2105810520420164, -343.8686284336190511 ) ) ;
#75807=CARTESIAN_POINT ( 'NONE',  ( -69.99304725725514231, -295.6443029165662324, -202.4472288391835946 ) ) ;
#75808=CARTESIAN_POINT ( 'NONE',  ( -36.19353185144915841, -283.0373591625779000, -343.3520880378246716 ) ) ;
#75809=CARTESIAN_POINT ( 'NONE',  ( -0.2649537176555840645, -275.9808626576804045, -206.7799908900141475 ) ) ;
#75810=CARTESIAN_POINT ( 'NONE',  ( 21.60523184260414808, -275.7491595865183172, -227.0268251121202923 ) ) ;
#75811=CARTESIAN_POINT ( 'NONE',  ( -22.10670906802912583, -284.8571383159976449, -343.7974556709527292 ) ) ;
#75812=ADVANCED_FACE ( 'NONE', ( #3797 ), #66578, .F. ) ;
#75813=CARTESIAN_POINT ( 'NONE',  ( -64.67130915957531556, -272.6070668355445719, -202.3231856295250282 ) ) ;
#75815=CARTESIAN_POINT ( 'NONE',  ( 204.1962367404059364, 292.3752467799872079, -53.99999999998791367 ) ) ;
#75816=CARTESIAN_POINT ( 'NONE',  ( 38.81623229397770558, -293.5275010491633338, -281.7175845855642251 ) ) ;
#75818=CARTESIAN_POINT ( 'NONE',  ( -98.87423496814145096, -285.9556975047948413, -312.7074508390106189 ) ) ;
#75820=CARTESIAN_POINT ( 'NONE',  ( -19.05039376806006857, -277.7666405000204577, -190.3683826091709363 ) ) ;
#75821=CARTESIAN_POINT ( 'NONE',  ( -28.62952085060375396, -276.1416396567680067, -346.7576007529440858 ) ) ;
#75822=CARTESIAN_POINT ( 'NONE',  ( -86.87997863990480596, -288.1275797692470633, -328.3303482179778143 ) ) ;
#75823=CARTESIAN_POINT ( 'NONE',  ( -81.02167324588612018, -285.1773066873630000, -329.7775032489919909 ) ) ;
#75824=CARTESIAN_POINT ( 'NONE',  ( -98.47333328313547440, -279.7397192771551317, -312.0851810841267593 ) ) ;
#75825=CARTESIAN_POINT ( 'NONE',  ( -35.18320931151639286, -287.5039888866168667, -193.9677946916732196 ) ) ;
#75826=CARTESIAN_POINT ( 'NONE',  ( -19.07134504114123885, -282.2873266987438683, -197.5668012903721547 ) ) ;
#75827=CARTESIAN_POINT ( 'NONE',  ( -68.84600606113829713, -273.8159883789961668, -200.0866435368874363 ) ) ;
#75828=CARTESIAN_POINT ( 'NONE',  ( -100.4667217371038390, -277.8025989422488919, -314.4545602543184373 ) ) ;
#75829=CARTESIAN_POINT ( 'NONE',  ( -58.80042892690541123, -297.2520488593347636, -341.6411092421834041 ) ) ;
#75831=EDGE_CURVE ( 'NONE', #53167, #1315, #90728, .T. ) ;
#75832=CARTESIAN_POINT ( 'NONE',  ( -69.85430415644619018, -279.9805209788416391, -337.9475929042657754 ) ) ;
#75833=CARTESIAN_POINT ( 'NONE',  ( -105.9189446312957159, -271.2171927607785165, -237.6329107657502107 ) ) ;
#75834=CARTESIAN_POINT ( 'NONE',  ( -35.12204278231480004, -276.5311816074056424, -343.3889316092275408 ) ) ;
#75835=CARTESIAN_POINT ( 'NONE',  ( -36.95721522690917737, -275.2619672315118464, -193.7461694587377110 ) ) ;
#75836=CARTESIAN_POINT ( 'NONE',  ( 33.23318227448275053, -289.0202663177749969, -248.0216449871566624 ) ) ;
#75837=CARTESIAN_POINT ( 'NONE',  ( -47.51976205650161944, -296.6994137995394567, -345.9859472841586694 ) ) ;
#75838=CARTESIAN_POINT ( 'NONE',  ( -36.26455936323313978, -296.2440359874659634, -346.9695094656361789 ) ) ;
#75839=CARTESIAN_POINT ( 'NONE',  ( 23.27516244509033427, -294.9531667750142105, -226.4574000748131084 ) ) ;
#75840=CARTESIAN_POINT ( 'NONE',  ( -60.27176484683163693, -277.7541595737312150, -199.0727770410573214 ) ) ;
#75841=CARTESIAN_POINT ( 'NONE',  ( 36.57259670622160996, -283.5920027569522972, -279.6134232125132826 ) ) ;
#75842=CARTESIAN_POINT ( 'NONE',  ( 53.90367334667526222, -297.2827687489743766, -195.9512618600769258 ) ) ;
#75843=CARTESIAN_POINT ( 'NONE',  ( -73.66267137309992563, -285.3889649012892278, -336.9109440597525804 ) ) ;
#75844=CARTESIAN_POINT ( 'NONE',  ( -10.62456063845134047, -285.3293322166863391, -202.0802608954608104 ) ) ;
#75845=CARTESIAN_POINT ( 'NONE',  ( 155.4712121400794445, 205.7503459434753381, -216.8500784743320651 ) ) ;
#75847=CARTESIAN_POINT ( 'NONE',  ( 11.15126855355469715, -286.4122628849373200, -215.6990439395227668 ) ) ;
#75849=CARTESIAN_POINT ( 'NONE',  ( -70.32466304100830712, -284.5563150361788871, -339.6114698006052208 ) ) ;
#75850=CARTESIAN_POINT ( 'NONE',  ( -19.27049385354924738, -274.6242924230606377, -199.5589839046129157 ) ) ;
#75851=CARTESIAN_POINT ( 'NONE',  ( 4.973188554968406727, -285.4048384834632657, -206.4429475523315602 ) ) ;
#75853=CARTESIAN_POINT ( 'NONE',  ( 23.55331173194532468, -281.8677609407910154, -223.5997537293674213 ) ) ;
#75855=CARTESIAN_POINT ( 'NONE',  ( -113.0319554170100815, -280.1995096954249789, -260.2788413600054582 ) ) ;
#75856=CARTESIAN_POINT ( 'NONE',  ( 39.25751857461231253, -281.9873993123113678, -278.5120697616152370 ) ) ;
#75857=CARTESIAN_POINT ( 'NONE',  ( 30.91033621190086578, -284.8380690714489560, -254.8156830097664738 ) ) ;
#75858=CARTESIAN_POINT ( 'NONE',  ( 198.2431558926663229, 284.9595988177349000, -111.8567102798726012 ) ) ;
#75860=CARTESIAN_POINT ( 'NONE',  ( 22.31345166405351677, -278.1716316210400350, -315.5417697541061557 ) ) ;
#75861=CARTESIAN_POINT ( 'NONE',  ( -90.79526613475253782, -229.9289224406445840, -347.4232527532336121 ) ) ;
#75862=CARTESIAN_POINT ( 'NONE',  ( 34.32058505444159380, -279.3020140620238294, -249.4717980706167850 ) ) ;
#75863=CARTESIAN_POINT ( 'NONE',  ( -1.168557828331867388, -296.3391519785228638, -337.2000398857312007 ) ) ;
#75864=CARTESIAN_POINT ( 'NONE',  ( -67.34462063162695245, -294.8049035803488778, -337.0360578957497069 ) ) ;
#75865=CARTESIAN_POINT ( 'NONE',  ( -110.3705018036671390, -290.3667222628482705, -245.9803694960368148 ) ) ;
#75867=CARTESIAN_POINT ( 'NONE',  ( -103.3317076770338474, -295.6331975501249758, -231.7351363714927857 ) ) ;
#75868=CARTESIAN_POINT ( 'NONE',  ( 30.14849459084241445, -286.3510009143491857, -300.3460609336086691 ) ) ;
#75869=CARTESIAN_POINT ( 'NONE',  ( 34.98414719972961962, -295.6302278905439493, -287.1455366750598728 ) ) ;
#75870=CARTESIAN_POINT ( 'NONE',  ( -49.51962599725477787, -287.2089537410172966, -197.8320898875983005 ) ) ;
#75872=CARTESIAN_POINT ( 'NONE',  ( 24.61743161434209526, -293.8898464370694228, -225.0412966328639470 ) ) ;
#75873=CARTESIAN_POINT ( 'NONE',  ( -108.9905448076058292, -285.2329558788666759, -256.0631636561234359 ) ) ;
#75874=CARTESIAN_POINT ( 'NONE',  ( -93.40936182729932113, -294.6317368279528068, -322.5764761156448799 ) ) ;
#75875=CARTESIAN_POINT ( 'NONE',  ( -98.89363678004025360, -290.7415144173950239, -316.3776322426410843 ) ) ;
#75876=CARTESIAN_POINT ( 'NONE',  ( -105.9520754209847837, -291.4944093431425358, -235.4277811038375603 ) ) ;
#75877=CARTESIAN_POINT ( 'NONE',  ( -53.40646254242511759, -289.4306940981847447, -341.5715344471017829 ) ) ;
#75880=CARTESIAN_POINT ( 'NONE',  ( -29.24840802400338902, -300.0128539397579175, -194.5937777933623352 ) ) ;
#75881=CARTESIAN_POINT ( 'NONE',  ( -38.33678194534609673, -272.8348684149425480, -193.7646524478022911 ) ) ;
#75882=CARTESIAN_POINT ( 'NONE',  ( 30.54817846180591090, -280.9775272945856841, -297.8269664604659965 ) ) ;
#75883=CARTESIAN_POINT ( 'NONE',  ( 4.834672031142612347, -274.1127332149424092, -205.9497839883548806 ) ) ;
#75884=CARTESIAN_POINT ( 'NONE',  ( -106.6457790048175838, -294.6996640615237197, -295.5642672307021144 ) ) ;
#75885=CARTESIAN_POINT ( 'NONE',  ( -39.16474588313371896, -278.9356897418955441, -344.5739335008564694 ) ) ;
#75886=CARTESIAN_POINT ( 'NONE',  ( 5.915415384517144659, -272.7848397515077181, -209.9677474299022606 ) ) ;
#75888=CARTESIAN_POINT ( 'NONE',  ( -60.65649446351395113, -298.9480649679464364, -200.7117299812641988 ) ) ;
#75889=CARTESIAN_POINT ( 'NONE',  ( -47.32840777196063442, -299.0020854215782720, -197.6839933183894686 ) ) ;
#75891=CARTESIAN_POINT ( 'NONE',  ( -111.5222636508694194, -297.9313295527707055, -287.8440360214779048 ) ) ;
#75893=CARTESIAN_POINT ( 'NONE',  ( -111.9128010852481196, -270.7153572753629760, -259.1636285309245977 ) ) ;
#75894=CARTESIAN_POINT ( 'NONE',  ( 23.02184643186814483, -294.7775512982865962, -311.6823437035922666 ) ) ;
#75895=CARTESIAN_POINT ( 'NONE',  ( 29.27961634384813294, -291.7066269868030304, -238.9841901662230157 ) ) ;
#75897=CARTESIAN_POINT ( 'NONE',  ( 31.19263554894574852, -275.5938141829099663, -235.3958246709615594 ) ) ;
#75898=CARTESIAN_POINT ( 'NONE',  ( -41.87389327199311140, -298.3267503824546338, -197.4807590913360400 ) ) ;
#75899=CIRCLE ( 'NONE', #15414, 3.038598599789554822 ) ;
#75900=CARTESIAN_POINT ( 'NONE',  ( 18.58020151246639529, -284.2335064384474208, -320.9463776469651179 ) ) ;
#75901=CARTESIAN_POINT ( 'NONE',  ( -8.242070812320026363, -281.3639406251772925, -341.1739835726905881 ) ) ;
#75902=CARTESIAN_POINT ( 'NONE',  ( -96.07671006737689368, -277.2309684685920956, -320.0152173543373237 ) ) ;
#75904=CARTESIAN_POINT ( 'NONE',  ( -109.1399280731205579, -283.5642832097281030, -284.4187205999521666 ) ) ;
#75905=CARTESIAN_POINT ( 'NONE',  ( -108.9470334338677304, -282.2570618757212060, -293.2663453970592400 ) ) ;
#75907=CARTESIAN_POINT ( 'NONE',  ( 28.55007982230936392, -274.5689972873958595, -303.2425081282113410 ) ) ;
#75908=CARTESIAN_POINT ( 'NONE',  ( -40.28239662771523655, -282.0154786147389814, -195.3686349565388127 ) ) ;
#75911=CARTESIAN_POINT ( 'NONE',  ( -43.95282829196552399, -272.3699124249708348, -194.3956945121152557 ) ) ;
#75912=CARTESIAN_POINT ( 'NONE',  ( -110.3124494798008044, -280.7840555670961180, -252.2722113796381791 ) ) ;
#75914=CARTESIAN_POINT ( 'NONE',  ( -92.36582407080817347, -285.7517920350217651, -322.1648260558247330 ) ) ;
#75916=CARTESIAN_POINT ( 'NONE',  ( 36.37296566227340122, -285.3710372959798178, -256.2661782117832558 ) ) ;
#75918=CARTESIAN_POINT ( 'NONE',  ( -92.49916027236018579, -294.6596093640908407, -318.7840990553311258 ) ) ;
#75919=CARTESIAN_POINT ( 'NONE',  ( -102.7423858827700229, -288.2194860516099766, -305.5930369968697278 ) ) ;
#75921=CARTESIAN_POINT ( 'NONE',  ( -57.55348217747368267, -284.2758537244203012, -196.7250779611132998 ) ) ;
#75922=CARTESIAN_POINT ( 'NONE',  ( 7.613689295216106601, -282.2770863868498168, -211.7690998939867768 ) ) ;
#75923=CARTESIAN_POINT ( 'NONE',  ( -11.07365303351870622, -280.9544067110335845, -341.7189313804644257 ) ) ;
#75924=CARTESIAN_POINT ( 'NONE',  ( -105.1130437040779100, -290.1874182480229933, -297.6269346142469772 ) ) ;
#75926=CARTESIAN_POINT ( 'NONE',  ( -92.66329760138118843, -280.6646627437276038, -221.8146746845749249 ) ) ;
#75927=CARTESIAN_POINT ( 'NONE',  ( -69.82116545691290810, -280.4159591185044178, -204.7905015080229418 ) ) ;
#75928=CARTESIAN_POINT ( 'NONE',  ( 29.94161605740303855, -289.0858619572676957, -236.4293900149949366 ) ) ;
#75930=CARTESIAN_POINT ( 'NONE',  ( -111.8182810546301198, -272.7992156270640862, -250.6061241805279565 ) ) ;
#75931=CARTESIAN_POINT ( 'NONE',  ( -110.3239333518953487, -292.7341566906680441, -254.6945791088535032 ) ) ;
#75933=CARTESIAN_POINT ( 'NONE',  ( -112.3417001280813849, -275.0519495502701943, -270.3929463913696054 ) ) ;
#75935=CARTESIAN_POINT ( 'NONE',  ( 37.72509889357520052, -273.4907655340558676, -265.5823357582788162 ) ) ;
#75937=CARTESIAN_POINT ( 'NONE',  ( -94.06977653310389087, -294.2543601270296563, -321.2565487766985370 ) ) ;
#75938=CARTESIAN_POINT ( 'NONE',  ( -91.19201809853579732, -272.6094591775613480, -220.9053986992230705 ) ) ;
#75939=CARTESIAN_POINT ( 'NONE',  ( -100.8921440408006447, -291.5635754280635865, -307.7717521966957861 ) ) ;
#75940=CARTESIAN_POINT ( 'NONE',  ( -26.57349754528888752, -284.6735780046901709, -343.6389456451801721 ) ) ;
#75941=CARTESIAN_POINT ( 'NONE',  ( -112.5948973674062330, -292.1444072122308171, -257.1111142486288372 ) ) ;
#75942=CARTESIAN_POINT ( 'NONE',  ( -3.554328762074253856, -293.8039260857265162, -201.7047652829031108 ) ) ;
#75943=CARTESIAN_POINT ( 'NONE',  ( 1.568037845835212662, -294.3498214268451534, -332.1869322365337212 ) ) ;
#75944=CARTESIAN_POINT ( 'NONE',  ( 5.857096093094018130, -288.6375055843107589, -208.9879991021803960 ) ) ;
#75945=CARTESIAN_POINT ( 'NONE',  ( 37.86598658131583051, -281.9261579276773091, -286.9387915925918833 ) ) ;
#75946=CARTESIAN_POINT ( 'NONE',  ( -111.2028154621348364, -294.4289458745433876, -286.2937839141118843 ) ) ;
#75947=CARTESIAN_POINT ( 'NONE',  ( -79.16150573856964456, -283.4330949595740776, -335.0148407152518075 ) ) ;
#75948=CARTESIAN_POINT ( 'NONE',  ( 30.66289900026975346, -277.9376964185632914, -301.1380784731194353 ) ) ;
#75949=CARTESIAN_POINT ( 'NONE',  ( -92.05005921254146983, -292.4090924074130839, -314.0302885647153062 ) ) ;
#75950=CARTESIAN_POINT ( 'NONE',  ( -111.5880219779992757, -276.4990930026191904, -285.5180161879386560 ) ) ;
#75953=CARTESIAN_POINT ( 'NONE',  ( -10.95939484926375052, -282.2064867201630136, -338.5466899743207705 ) ) ;
#75955=CARTESIAN_POINT ( 'NONE',  ( -108.1514886672800060, -280.1305568707308566, -241.1381379045861308 ) ) ;
#75956=CARTESIAN_POINT ( 'NONE',  ( 0.1792849999216633017, -285.5978368967813594, -203.3760033283395501 ) ) ;
#75957=CARTESIAN_POINT ( 'NONE',  ( 33.59391552437426043, -295.0345133766168715, -249.0633222129276874 ) ) ;
#75958=CARTESIAN_POINT ( 'NONE',  ( 38.90709530625224488, -277.1621598068036292, -271.1428842655080302 ) ) ;
#75960=CARTESIAN_POINT ( 'NONE',  ( 38.25117004177573676, -277.0199203808313086, -282.4845915570071497 ) ) ;
#75961=CARTESIAN_POINT ( 'NONE',  ( -39.15989041254362490, -276.9089216448539332, -343.3384719262245994 ) ) ;
#75962=CARTESIAN_POINT ( 'NONE',  ( -33.72611932015692560, -300.0976701652980978, -195.5265398058162702 ) ) ;
#75963=CARTESIAN_POINT ( 'NONE',  ( -107.2692529344595869, -282.8990944411660848, -243.7121821111891222 ) ) ;
#75965=CARTESIAN_POINT ( 'NONE',  ( -53.38076770319752029, -291.5187051769832465, -195.0172433845634714 ) ) ;
#75966=CARTESIAN_POINT ( 'NONE',  ( -96.65439090270751876, -291.5040083434977305, -318.2193847732332870 ) ) ;
#75968=CARTESIAN_POINT ( 'NONE',  ( 2.419655016270580994, -291.5187664587163567, -208.7115247410452241 ) ) ;
#75970=CARTESIAN_POINT ( 'NONE',  ( -56.02699608372067530, -290.3909448486285214, -196.2156633963072068 ) ) ;
#75971=CARTESIAN_POINT ( 'NONE',  ( 33.32973783826315639, -292.9763526627592114, -251.9862617214188560 ) ) ;
#75973=CARTESIAN_POINT ( 'NONE',  ( -104.8772340428890004, -291.1600957520788029, -306.6990343754949322 ) ) ;
#75974=CARTESIAN_POINT ( 'NONE',  ( -76.88395952052188420, -280.1589448643318860, -208.8166071297662256 ) ) ;
#75976=CARTESIAN_POINT ( 'NONE',  ( -113.3481868144358060, -295.3392275439289278, -280.9734097568272091 ) ) ;
#75977=CARTESIAN_POINT ( 'NONE',  ( 0.2267371477746556729, -287.1902449482997781, -203.2497028568727160 ) ) ;
#75978=CARTESIAN_POINT ( 'NONE',  ( 36.76521087307970959, -288.1470900618989504, -291.2399758316909129 ) ) ;
#75979=CARTESIAN_POINT ( 'NONE',  ( -84.87232902196633688, -284.0625601656288381, -325.7951039806498557 ) ) ;
#75980=CARTESIAN_POINT ( 'NONE',  ( -90.36657093633624527, -230.3778195935935003, -347.8114039112169849 ) ) ;
#75981=CARTESIAN_POINT ( 'NONE',  ( -85.04316653643064683, -218.3528564987888103, -351.0001102442844285 ) ) ;
#75982=CARTESIAN_POINT ( 'NONE',  ( 138.1549688690315918, 178.5493954107672039, -238.2378617337843139 ) ) ;
#75983=CARTESIAN_POINT ( 'NONE',  ( 33.66837277626137137, -274.5174278050423027, -252.7494379492692929 ) ) ;
#75984=CARTESIAN_POINT ( 'NONE',  ( 35.66058051292321096, -274.5604895844408020, -277.0613488986852531 ) ) ;
#75985=CARTESIAN_POINT ( 'NONE',  ( -110.7525165698548051, -296.3514061935542827, -247.1546002169693566 ) ) ;
#75986=CARTESIAN_POINT ( 'NONE',  ( 174.8086493686545566, 240.3597952296187827, -177.5534806918111883 ) ) ;
#75987=CARTESIAN_POINT ( 'NONE',  ( 35.58745166541468308, -274.5294829806975940, -293.4833387096866204 ) ) ;
#75988=CARTESIAN_POINT ( 'NONE',  ( -72.40733836790208500, -275.3419526731543101, -205.1244447376594735 ) ) ;
#75989=CARTESIAN_POINT ( 'NONE',  ( -20.58583114906167566, -299.1983710257756570, -193.5938057002267385 ) ) ;
#75990=CARTESIAN_POINT ( 'NONE',  ( -75.89589603595813116, -290.0746458086439361, -332.4220752706754638 ) ) ;
#75991=CARTESIAN_POINT ( 'NONE',  ( -107.0156433830699996, -296.9394437326857314, -302.7601990080789278 ) ) ;
#75992=CARTESIAN_POINT ( 'NONE',  ( -111.5643769034880819, -297.3006958774917052, -249.9028719166121846 ) ) ;
#75993=CARTESIAN_POINT ( 'NONE',  ( -34.29907000615826007, -295.1795156242868075, -343.2976822453702539 ) ) ;
#75994=ORIENTED_EDGE ( 'NONE', *, *, #4077, .F. ) ;
#75995=CARTESIAN_POINT ( 'NONE',  ( 7.408287121446841539, -278.3678564565182114, -331.3090201194807491 ) ) ;
#75997=CARTESIAN_POINT ( 'NONE',  ( -17.00222038531473245, -279.8156233805706279, -196.1598210473968891 ) ) ;
#75998=CARTESIAN_POINT ( 'NONE',  ( -83.14460891177755286, -278.6381134529114547, -327.5709484809809169 ) ) ;
#75999=CARTESIAN_POINT ( 'NONE',  ( -53.88846030834669421, -279.0217260709594029, -344.5782259279454252 ) ) ;
#76000=CARTESIAN_POINT ( 'NONE',  ( -38.54454208212246158, -275.0872776358256147, -345.7067215570374401 ) ) ;
#76001=CARTESIAN_POINT ( 'NONE',  ( -74.30992935990809656, -274.0390524495335853, -207.2839531359876446 ) ) ;
#76003=CARTESIAN_POINT ( 'NONE',  ( -84.43812335347153919, -295.9640594180127664, -213.7499117009384406 ) ) ;
#76005=CARTESIAN_POINT ( 'NONE',  ( -108.1715647033971806, -278.4850744267726554, -288.0798524474452051 ) ) ;
#76006=CARTESIAN_POINT ( 'NONE',  ( -24.19730974589690575, -275.0185951405136962, -194.6011629654353783 ) ) ;
#76007=CARTESIAN_POINT ( 'NONE',  ( -57.17928305227649588, -287.9875900632906678, -344.3061206459876757 ) ) ;
#76008=CARTESIAN_POINT ( 'NONE',  ( -43.89409087027367207, -275.9696206021974945, -195.5959630775169558 ) ) ;
#76010=CARTESIAN_POINT ( 'NONE',  ( -63.88900274588976913, -288.6044308017839626, -338.5905129820301340 ) ) ;
#76011=CARTESIAN_POINT ( 'NONE',  ( -80.87366006422885789, -284.8271148757268634, -206.9069346341300957 ) ) ;
#76012=CARTESIAN_POINT ( 'NONE',  ( 20.12483232928461163, -280.4431770220854787, -317.0241118479720512 ) ) ;
#76013=CARTESIAN_POINT ( 'NONE',  ( 18.93331755614955725, -280.7953119192370082, -317.7989952549624491 ) ) ;
#76014=CARTESIAN_POINT ( 'NONE',  ( -30.37258982855084000, -284.2206814078384696, -196.1962563974661862 ) ) ;
#76015=CARTESIAN_POINT ( 'NONE',  ( -0.9407073142919682995, -290.5694564146256766, -335.9927982852373702 ) ) ;
#76016=CARTESIAN_POINT ( 'NONE',  ( -104.8130807538472027, -280.1432436811634261, -241.4691935017444564 ) ) ;
#76019=CARTESIAN_POINT ( 'NONE',  ( -40.57244151061917847, -294.0117071832756324, -195.4178909076942432 ) ) ;
#76020=CARTESIAN_POINT ( 'NONE',  ( -111.9963532124225623, -276.9724159568884261, -256.1262997992009787 ) ) ;
#76022=CARTESIAN_POINT ( 'NONE',  ( -11.20986616441890504, -277.3537986155270687, -338.6327806393072706 ) ) ;
#76023=CARTESIAN_POINT ( 'NONE',  ( -101.3434009962186479, -286.0245128532798162, -309.7795237229511258 ) ) ;
#76024=EDGE_CURVE ( 'NONE', #53167, #69774, #37829, .T. ) ;
#76027=DIRECTION ( 'NONE',  ( 0.000000000000000000, 0.000000000000000000, 1.000000000000000000 ) ) ;
#76028=CARTESIAN_POINT ( 'NONE',  ( -67.45705456184020932, -291.3642470151970656, -339.6603216404498085 ) ) ;
#76030=CARTESIAN_POINT ( 'NONE',  ( -110.3465916710653545, -294.3307108219991051, -287.5999104957114128 ) ) ;
#76031=CARTESIAN_POINT ( 'NONE',  ( 38.51389189407272085, -286.9069115583802159, -282.9353773197545365 ) ) ;
#76032=CARTESIAN_POINT ( 'NONE',  ( -75.37460983632033162, -289.9361834806989577, -207.0564003974298544 ) ) ;
#76034=CARTESIAN_POINT ( 'NONE',  ( 19.55279810706876020, -274.8914941718879277, -316.9025458673040703 ) ) ;
#76035=CARTESIAN_POINT ( 'NONE',  ( -71.52023349363894056, -293.6481243479290129, -336.2744556876218667 ) ) ;
#76038=CARTESIAN_POINT ( 'NONE',  ( -113.5597172241179038, -288.9856254112971214, -274.0382936655008166 ) ) ;
#76039=CARTESIAN_POINT ( 'NONE',  ( -69.13787289579103401, -287.2269187639383858, -203.7480474070543153 ) ) ;
#76040=CARTESIAN_POINT ( 'NONE',  ( -9.949808324987175823, -286.9391682151593841, -341.2388879613669133 ) ) ;
#76041=CARTESIAN_POINT ( 'NONE',  ( -108.9948986926918622, -285.7573339169599080, -287.1849568370683983 ) ) ;
#76043=CARTESIAN_POINT ( 'NONE',  ( -42.69612697970789839, -286.7857398359332137, -197.3831861166171677 ) ) ;
#76044=CARTESIAN_POINT ( 'NONE',  ( 37.96410137081927871, -295.5669115517113141, -273.0893152886368398 ) ) ;
#76045=CARTESIAN_POINT ( 'NONE',  ( -69.70683069490866046, -275.5546957679982256, -338.6527543176570703 ) ) ;
#76046=CARTESIAN_POINT ( 'NONE',  ( -106.3245471169879579, -278.4448854882502360, -304.6440419186031932 ) ) ;
#76047=CARTESIAN_POINT ( 'NONE',  ( 34.91718699693180383, -291.3493499639941433, -248.2711331495324885 ) ) ;
#76048=CARTESIAN_POINT ( 'NONE',  ( -35.11085582536794192, -300.0601007652616659, -195.7155521100123963 ) ) ;
#76050=CARTESIAN_POINT ( 'NONE',  ( -110.9470825032862820, -282.3671488964955074, -284.7572402772948976 ) ) ;
#76052=CARTESIAN_POINT ( 'NONE',  ( -105.5681333782994074, -277.0782454512280992, -241.1033107563759756 ) ) ;
#76053=CARTESIAN_POINT ( 'NONE',  ( 30.57030059763306795, -279.9718200200854312, -302.3104308716163473 ) ) ;
#76055=CARTESIAN_POINT ( 'NONE',  ( 14.39871299181071862, -274.8205415338319426, -326.5189986597804364 ) ) ;
#76056=CARTESIAN_POINT ( 'NONE',  ( -105.5968602864647323, -297.7035912348071065, -298.1449417418108965 ) ) ;
#76058=CARTESIAN_POINT ( 'NONE',  ( -35.91877279613662211, -281.9550661235056737, -347.0518701350185324 ) ) ;
#76059=CARTESIAN_POINT ( 'NONE',  ( -72.97180650640677868, -298.5088205713158800, -206.3774953287440326 ) ) ;
#76060=CARTESIAN_POINT ( 'NONE',  ( -91.29966478901761207, -298.6191288769531411, -216.1224203418156549 ) ) ;
#76061=CARTESIAN_POINT ( 'NONE',  ( -67.06222564507206130, -273.3182351341887397, -203.6482622081232705 ) ) ;
#76062=CARTESIAN_POINT ( 'NONE',  ( 37.70948608006271741, -295.5572517172814173, -270.7454272195612930 ) ) ;
#76063=CARTESIAN_POINT ( 'NONE',  ( 35.07319506592877900, -288.0511312081731603, -296.6903482713996709 ) ) ;
#76064=CARTESIAN_POINT ( 'NONE',  ( 30.73485323614489317, -274.1270672462239872, -303.7354388363376643 ) ) ;
#76065=CARTESIAN_POINT ( 'NONE',  ( 16.68444365934453799, -288.1427482256304415, -325.3003286409004318 ) ) ;
#76066=CARTESIAN_POINT ( 'NONE',  ( 14.24063675421330899, -287.3639591154873187, -322.3483372739083848 ) ) ;
#76067=CARTESIAN_POINT ( 'NONE',  ( -112.1206062431190702, -288.4698658283209056, -276.7570070170708618 ) ) ;
#76068=ORIENTED_EDGE ( 'NONE', *, *, #46451, .F. ) ;
#76069=CARTESIAN_POINT ( 'NONE',  ( 168.1488725781630649, 234.1813984995739588, -193.4213935641190858 ) ) ;
#76070=CARTESIAN_POINT ( 'NONE',  ( 24.28689484107245278, -287.6019351796898036, -309.6027377726563259 ) ) ;
#76072=CARTESIAN_POINT ( 'NONE',  ( -106.4724330804543371, -285.9228948723415442, -236.9880453978409776 ) ) ;
#76073=CARTESIAN_POINT ( 'NONE',  ( -4.693298396127183025, -291.5305477319059264, -200.8852079244021240 ) ) ;
#76074=CARTESIAN_POINT ( 'NONE',  ( 10.30672033035423141, -282.2968452250051996, -210.8286512880796408 ) ) ;
#76075=CARTESIAN_POINT ( 'NONE',  ( -6.444976512106915578, -281.7646787273274640, -200.3562913039808961 ) ) ;
#76076=CARTESIAN_POINT ( 'NONE',  ( -56.32094479663410169, -283.1369305463718433, -340.8507503854584684 ) ) ;
#76077=CARTESIAN_POINT ( 'NONE',  ( 15.14878992875681796, -278.3119622101590949, -324.0035116118828000 ) ) ;
#76078=CARTESIAN_POINT ( 'NONE',  ( -110.7997946007286316, -296.2615738536190406, -293.4900583394814930 ) ) ;
#76079=CARTESIAN_POINT ( 'NONE',  ( -108.4213384445573780, -274.1146472706962527, -251.4861789237028518 ) ) ;
#76080=CARTESIAN_POINT ( 'NONE',  ( -70.93895424918967763, -289.6266879276687405, -203.7047505313932447 ) ) ;
#76081=CARTESIAN_POINT ( 'NONE',  ( -110.2786492092206885, -271.4547307310580777, -262.1555123849296933 ) ) ;
#76084=CARTESIAN_POINT ( 'NONE',  ( -110.6147194032072605, -286.6430841782876655, -257.1599668740173001 ) ) ;
#76086=CARTESIAN_POINT ( 'NONE',  ( -61.48117441133690164, -296.4380729176240266, -343.2093368443427721 ) ) ;
#76087=CARTESIAN_POINT ( 'NONE',  ( -107.0806176643818191, -284.9134692792322312, -292.2786007098782761 ) ) ;
#76088=CARTESIAN_POINT ( 'NONE',  ( 39.39597081608347651, -274.5853459679027537, -268.3239458345869366 ) ) ;
#76089=CARTESIAN_POINT ( 'NONE',  ( -70.86078524371089316, -292.2728980964574248, -201.1528546015402696 ) ) ;
#76090=CARTESIAN_POINT ( 'NONE',  ( -107.8698363859662095, -283.0499521734768678, -242.5402707553669472 ) ) ;
#76091=CARTESIAN_POINT ( 'NONE',  ( -2.069309449261933942, -292.8394817343975660, -201.9241060530037544 ) ) ;
#76093=CARTESIAN_POINT ( 'NONE',  ( -34.57294953326663034, -289.3498277015729627, -343.3793475435304003 ) ) ;
#76095=AXIS2_PLACEMENT_3D ( 'NONE', #28969, #86708, #21873 ) ;
#76097=CARTESIAN_POINT ( 'NONE',  ( 6.451691864244251562, -59.65713888448967595, -351.0909003801652375 ) ) ;
#76098=CARTESIAN_POINT ( 'NONE',  ( -113.2124118153363810, -285.9694803670265060, -278.5062306186741239 ) ) ;
#76099=CARTESIAN_POINT ( 'NONE',  ( -95.99890600148557951, -293.4094976428775681, -317.0979686699210447 ) ) ;
#76101=CARTESIAN_POINT ( 'NONE',  ( 17.30236139984067378, -279.7762853634818612, -221.4913664608390036 ) ) ;
#76102=CARTESIAN_POINT ( 'NONE',  ( 5.855908976923163145, -276.1504848360327173, -334.0769783241346431 ) ) ;
#76103=CARTESIAN_POINT ( 'NONE',  ( -106.1372464149112886, -280.9382004354164337, -240.9128373064592381 ) ) ;
#76104=CARTESIAN_POINT ( 'NONE',  ( 27.36103610868812908, -24.54272754578916249, -343.3512226634238687 ) ) ;
#76105=CARTESIAN_POINT ( 'NONE',  ( -44.38313441369549395, -281.7141632033985843, -346.4997068946032073 ) ) ;
#76106=CARTESIAN_POINT ( 'NONE',  ( -110.5984609935359089, -282.3874139172017408, -284.6891950701244127 ) ) ;
#76108=CARTESIAN_POINT ( 'NONE',  ( -98.58286273371544439, -275.0152257852059847, -225.6666292473326223 ) ) ;
#76109=CARTESIAN_POINT ( 'NONE',  ( -68.53792374930726794, -295.9657901631740060, -336.4413729006775498 ) ) ;
#76111=CARTESIAN_POINT ( 'NONE',  ( 35.91466781810470366, -292.3142112879884280, -276.2558641556560133 ) ) ;
#76112=CARTESIAN_POINT ( 'NONE',  ( 38.08401046024775383, -276.3911036465935354, -285.3369307880264500 ) ) ;
#76113=CARTESIAN_POINT ( 'NONE',  ( -29.98986665155448250, -274.1477929672778941, -197.7322632171610053 ) ) ;
#76114=CARTESIAN_POINT ( 'NONE',  ( 22.52571284700371379, -273.8276629161189248, -222.4092399869006442 ) ) ;
#76116=CARTESIAN_POINT ( 'NONE',  ( -4.249203765795510179, -272.4881347513623950, -203.0426458878170308 ) ) ;
#76120=CARTESIAN_POINT ( 'NONE',  ( 12.13539671357389693, -283.4238804594296539, -324.4558770727243200 ) ) ;
#76121=CARTESIAN_POINT ( 'NONE',  ( -3.326083706890943681, -284.3694042368343844, -338.3234414275487438 ) ) ;
#76122=CARTESIAN_POINT ( 'NONE',  ( -110.0950005561461751, -284.0012465296653090, -262.7311777370776440 ) ) ;
#76123=CARTESIAN_POINT ( 'NONE',  ( -32.38698326070905864, -275.3886508705768392, -344.0451246684216926 ) ) ;
#76124=CARTESIAN_POINT ( 'NONE',  ( 30.45199406605279080, -283.8145644404988843, -300.7344161441818073 ) ) ;
#76125=CARTESIAN_POINT ( 'NONE',  ( -54.13052162131204881, -275.7513924861306123, -342.1691973884592244 ) ) ;
#76126=CARTESIAN_POINT ( 'NONE',  ( -1.583818916418291423, -275.6176602082504132, -206.3498702297087846 ) ) ;
#76128=CARTESIAN_POINT ( 'NONE',  ( -56.52624197746927592, -280.6139448484572654, -195.9011761911354199 ) ) ;
#76132=CARTESIAN_POINT ( 'NONE',  ( -109.0478871218274719, -286.0992788355792982, -294.8259545129931212 ) ) ;
#76133=CARTESIAN_POINT ( 'NONE',  ( -7.932760715127213480, -293.8538909085236241, -337.3651416634506290 ) ) ;
#76134=CARTESIAN_POINT ( 'NONE',  ( -114.0115551577167992, -289.8183958810299146, -276.9366082656763979 ) ) ;
#76135=CARTESIAN_POINT ( 'NONE',  ( 26.55978144643145100, -286.2987876544191863, -307.8063924156029429 ) ) ;
#76136=CARTESIAN_POINT ( 'NONE',  ( -6.755171173920111016, -285.0364444681046052, -203.4156778648855379 ) ) ;
#76137=CARTESIAN_POINT ( 'NONE',  ( -66.94913751108470024, -289.8985505982098516, -202.5276921000277923 ) ) ;
#76138=CARTESIAN_POINT ( 'NONE',  ( -93.71725922283104637, -285.0939094030924252, -317.3603397071559584 ) ) ;
#76139=CARTESIAN_POINT ( 'NONE',  ( -8.673318798625839321, -274.6768893177790005, -339.6796075054556923 ) ) ;
#76140=CARTESIAN_POINT ( 'NONE',  ( 30.71651624715849138, -285.5064175604962315, -236.0898530914087985 ) ) ;
#76141=CARTESIAN_POINT ( 'NONE',  ( -32.11032877462433532, -300.1177950843049302, -195.3593257338152114 ) ) ;
#76142=CARTESIAN_POINT ( 'NONE',  ( 13.03747359438205322, -284.7533051515300713, -214.5062549990608147 ) ) ;
#76143=CARTESIAN_POINT ( 'NONE',  ( 11.45370304120203464, -281.6901796690403899, -215.7496075011398773 ) ) ;
#76144=CARTESIAN_POINT ( 'NONE',  ( -79.49100149355670908, -291.6197162158988476, -332.6611486431770572 ) ) ;
#76148=CARTESIAN_POINT ( 'NONE',  ( -39.05030000327838025, -296.9935862307967795, -345.9018016420998265 ) ) ;
#76149=CARTESIAN_POINT ( 'NONE',  ( -0.9745784581178658090, -278.5348183059059579, -204.7681830609684255 ) ) ;
#76150=CARTESIAN_POINT ( 'NONE',  ( -5.943545222788352511, -291.6516268500353704, -200.2161613024450162 ) ) ;
#76151=CARTESIAN_POINT ( 'NONE',  ( -111.1848895209751049, -294.9377440495641167, -271.4548583908583623 ) ) ;
#76152=CARTESIAN_POINT ( 'NONE',  ( 22.98003335751389997, -280.8182271328700494, -312.3436375328074632 ) ) ;
#76153=CARTESIAN_POINT ( 'NONE',  ( 10.42751909942468913, -272.7969640136547014, -213.2023037157763667 ) ) ;
#76154=CARTESIAN_POINT ( 'NONE',  ( 35.32816335982330713, -295.0154124352441158, -281.6623330039305984 ) ) ;
#76155=CARTESIAN_POINT ( 'NONE',  ( -4.829096099716510437, -294.9805209788416391, -202.7746430608542312 ) ) ;
#76156=CARTESIAN_POINT ( 'NONE',  ( -111.8645635446429054, -271.3396278418827592, -253.4806818537858533 ) ) ;
#76157=CARTESIAN_POINT ( 'NONE',  ( -19.54662964627135935, -293.0663389252223965, -344.2888823901656110 ) ) ;
#76159=CARTESIAN_POINT ( 'NONE',  ( 9.207639428972127504, -294.1309697270799575, -213.2991249091605255 ) ) ;
#76161=CARTESIAN_POINT ( 'NONE',  ( 33.60514948766985555, -294.5902378573332498, -288.2257830242676846 ) ) ;
#76163=CARTESIAN_POINT ( 'NONE',  ( -55.33440940062592972, -281.3026256464106041, -343.5367232947555749 ) ) ;
#76164=CARTESIAN_POINT ( 'NONE',  ( -15.59282841151147458, -294.7628665931050023, -340.0991984537363351 ) ) ;
#76166=CARTESIAN_POINT ( 'NONE',  ( 36.47868067795234026, -281.8289688222096743, -292.4432063663202257 ) ) ;
#76167=CARTESIAN_POINT ( 'NONE',  ( -110.6667003585914415, -283.9236722787348981, -293.8393690874095796 ) ) ;
#76168=CARTESIAN_POINT ( 'NONE',  ( -53.83681850528533630, -287.2642022859209305, -343.3538538751236047 ) ) ;
#76170=CARTESIAN_POINT ( 'NONE',  ( -10.96007420478843741, -281.1943872675498710, -342.0183486038312708 ) ) ;
#76172=CARTESIAN_POINT ( 'NONE',  ( 7.741645972113681218, -287.3732558840783327, -332.4667810086199893 ) ) ;
#76174=CARTESIAN_POINT ( 'NONE',  ( -2.750946930590558726, -296.1869150250240637, -335.5525300693781219 ) ) ;
#76175=CARTESIAN_POINT ( 'NONE',  ( -12.04400716799281490, -278.1546641365202390, -342.5181689210476748 ) ) ;
#76176=CARTESIAN_POINT ( 'NONE',  ( -108.3092153509391835, -278.4456849880803020, -253.1652094586677038 ) ) ;
#76177=CARTESIAN_POINT ( 'NONE',  ( -13.86847411476865943, -292.5150805279670294, -196.9702428282546123 ) ) ;
#76179=CARTESIAN_POINT ( 'NONE',  ( -13.89247716168959101, -280.8300564381304412, -342.1904165909267590 ) ) ;
#76181=CARTESIAN_POINT ( 'NONE',  ( 34.18218954774205542, -292.4031678975247814, -254.5632775188253447 ) ) ;
#76182=CARTESIAN_POINT ( 'NONE',  ( -108.8994442186181857, -294.2617360929501160, -292.8650043882645377 ) ) ;
#76186=CARTESIAN_POINT ( 'NONE',  ( 33.17444996187899875, -293.3126895032967809, -289.5257052011448877 ) ) ;
#76188=CARTESIAN_POINT ( 'NONE',  ( 17.36665895637873192, -291.6952119285918457, -314.0302885647153062 ) ) ;
#76189=CARTESIAN_POINT ( 'NONE',  ( -31.91811639151086766, -297.1772509278766847, -193.5972525813361074 ) ) ;
#76190=CARTESIAN_POINT ( 'NONE',  ( 30.91907146842683218, -279.2617524575707648, -237.3652354966351083 ) ) ;
#76191=CARTESIAN_POINT ( 'NONE',  ( 33.39702184604652047, -288.4930101215028913, -241.0794989330513260 ) ) ;
#76192=CARTESIAN_POINT ( 'NONE',  ( -5.794353780739670334, -288.4587008117282494, -336.1924550719858189 ) ) ;
#76193=CARTESIAN_POINT ( 'NONE',  ( -73.16224152467334818, -279.0562693167220800, -334.7774711732768083 ) ) ;
#76194=CARTESIAN_POINT ( 'NONE',  ( -40.58449608220404770, -299.7709930978458033, -196.4061319642943602 ) ) ;
#76196=CARTESIAN_POINT ( 'NONE',  ( -78.86923746328997709, -276.4203335142410083, -330.9423841821011933 ) ) ;
#76198=CARTESIAN_POINT ( 'NONE',  ( -80.60962900258410002, -297.1499246020748046, -206.6289016264463498 ) ) ;
#76199=CARTESIAN_POINT ( 'NONE',  ( -74.23786127341048768, -291.4667465931088941, -335.0286341508721080 ) ) ;
#76200=CARTESIAN_POINT ( 'NONE',  ( 38.85525595660539722, -295.1154479318924473, -267.4466598667569883 ) ) ;
#76202=CARTESIAN_POINT ( 'NONE',  ( -86.79223756958316471, -290.4129738191232946, -324.2678437636218973 ) ) ;
#76204=CARTESIAN_POINT ( 'NONE',  ( -110.7183655319142019, -297.4949820912572136, -247.1806778513567053 ) ) ;
#76205=CARTESIAN_POINT ( 'NONE',  ( -105.4143060338692663, -288.2562895974788830, -303.7434260337585670 ) ) ;
#76206=CARTESIAN_POINT ( 'NONE',  ( -75.77303195036481043, -297.8874081006112533, -203.6007872815017947 ) ) ;
#76208=DIRECTION ( 'NONE',  ( -1.000000000000000000, -0.000000000000000000, -0.000000000000000000 ) ) ;
#76209=CARTESIAN_POINT ( 'NONE',  ( -99.47782662320248903, -292.6642216147709519, -226.0687988101013559 ) ) ;
#76210=CARTESIAN_POINT ( 'NONE',  ( 36.60358173371528068, -296.4805209788416391, -305.9350535429201159 ) ) ;
#76211=CARTESIAN_POINT ( 'NONE',  ( -72.05061536490396179, -287.5921755817422536, -204.0639111605298694 ) ) ;
#76212=CARTESIAN_POINT ( 'NONE',  ( -21.52224098468846236, -272.2552977652755999, -197.2189746191602921 ) ) ;
#76213=CARTESIAN_POINT ( 'NONE',  ( -54.56804387304662640, -275.7492352321035014, -197.9417333119921807 ) ) ;
#76214=CARTESIAN_POINT ( 'NONE',  ( -109.8241076460055439, -288.8521103906546728, -253.3463959635021752 ) ) ;
#76215=CARTESIAN_POINT ( 'NONE',  ( -67.19966758303387167, -279.2998936537179588, -339.9944954805196176 ) ) ;
#76216=CARTESIAN_POINT ( 'NONE',  ( -43.75108986543212808, -279.9690414437212667, -197.5928001481529463 ) ) ;
#76217=CARTESIAN_POINT ( 'NONE',  ( -61.57632958888007124, -282.7239422256514558, -339.3823613209391965 ) ) ;
#76218=CARTESIAN_POINT ( 'NONE',  ( -42.77051135094828282, -278.1988168739889034, -346.8596180892677125 ) ) ;
#76219=CARTESIAN_POINT ( 'NONE',  ( 32.81546619092550543, -279.9528151303060781, -239.6043182205529263 ) ) ;
#76220=CARTESIAN_POINT ( 'NONE',  ( 151.9403889390961240, 205.9175150728080439, -214.8626715079458904 ) ) ;
#76221=CARTESIAN_POINT ( 'NONE',  ( 1.067278298569687367, -275.4929940158611998, -203.8810736652323783 ) ) ;
#76223=CARTESIAN_POINT ( 'NONE',  ( -91.68896306329104107, -274.8146490932733741, -216.7972984447000329 ) ) ;
#76224=CARTESIAN_POINT ( 'NONE',  ( 7.399455738971494334, -277.1948066931273047, -214.2051214447836571 ) ) ;
#76228=CARTESIAN_POINT ( 'NONE',  ( 22.22083613111720979, -289.2267314906696924, -313.0990443304157225 ) ) ;
#76229=CARTESIAN_POINT ( 'NONE',  ( 6.935038215161405617, -288.4053908461635842, -208.5424231130983799 ) ) ;
#76230=CARTESIAN_POINT ( 'NONE',  ( -80.47432844673046759, -289.0025470480873082, -329.4450335138739092 ) ) ;
#76231=CARTESIAN_POINT ( 'NONE',  ( 22.04667438303508575, -286.4021073552116832, -221.4474401773227328 ) ) ;
#76233=CARTESIAN_POINT ( 'NONE',  ( 12.44149653315743542, -280.7445121722610111, -324.8411486703859055 ) ) ;
#76234=CARTESIAN_POINT ( 'NONE',  ( 29.34762096092801187, -289.8469195111678687, -302.9709313845942802 ) ) ;
#76235=CARTESIAN_POINT ( 'NONE',  ( -68.09115084047047617, -281.9433191321730874, -337.3325972496724034 ) ) ;
#76236=CARTESIAN_POINT ( 'NONE',  ( -110.1125250017011581, -280.0066481343555438, -259.7287960100724717 ) ) ;
#76238=CARTESIAN_POINT ( 'NONE',  ( -24.31247500908635573, -277.3737919798914504, -342.3029996870943137 ) ) ;
#76239=CARTESIAN_POINT ( 'NONE',  ( -100.3627047681104187, -288.7690257045032922, -313.9083531752284557 ) ) ;
#76240=CARTESIAN_POINT ( 'NONE',  ( -87.65195034795991091, -286.1735348565533172, -212.2128125754102825 ) ) ;
#76241=CARTESIAN_POINT ( 'NONE',  ( 22.93975552307198029, -287.4039946583444589, -222.5314088620413600 ) ) ;
#76242=CARTESIAN_POINT ( 'NONE',  ( -40.23223348366850161, -283.2561758089654518, -343.3038682833472990 ) ) ;
#76245=CARTESIAN_POINT ( 'NONE',  ( -81.23438751810218150, -293.3229321674481298, -208.6056528654344504 ) ) ;
#76247=CARTESIAN_POINT ( 'NONE',  ( 10.87445188436011279, -293.0863395316068818, -329.8305635953509523 ) ) ;
#76248=AXIS2_PLACEMENT_3D ( 'NONE', #18571, #69703, #83901 ) ;
#76249=CARTESIAN_POINT ( 'NONE',  ( 0.7450351216454592640, -273.6324716830128523, -207.8086676223443874 ) ) ;
#76250=EDGE_CURVE ( 'NONE', #44141, #46969, #46845, .T. ) ;
#76251=CARTESIAN_POINT ( 'NONE',  ( -19.31923069674204285, -294.1748885325274045, -345.1722228434732642 ) ) ;
#76252=CARTESIAN_POINT ( 'NONE',  ( -77.61805655244667435, -289.9804857328609842, -208.6478871105687176 ) ) ;
#76253=CARTESIAN_POINT ( 'NONE',  ( -63.95399614429018698, -293.6437524977787916, -339.4788744237098967 ) ) ;
#76254=CARTESIAN_POINT ( 'NONE',  ( -71.34314728681985684, -290.7166507677868026, -335.4217002395019449 ) ) ;
#76256=TOROIDAL_SURFACE ( 'NONE', #92873, 5.654241149514405151, 1.000000000000000000 ) ;
#76257=CARTESIAN_POINT ( 'NONE',  ( -4.108406303805257842, -290.4891287321794948, -202.9260320208372832 ) ) ;
#76258=CARTESIAN_POINT ( 'NONE',  ( 28.48397989213211545, -295.0734138936728641, -234.3103449144501553 ) ) ;
#76259=CARTESIAN_POINT ( 'NONE',  ( 22.95040097869604523, -289.0707723354784093, -311.9557063478078476 ) ) ;
#76260=CARTESIAN_POINT ( 'NONE',  ( 34.99957049443172963, -277.2595651719407783, -249.0804711168652830 ) ) ;
#76261=CARTESIAN_POINT ( 'NONE',  ( -28.66135202697728346, -275.7394613280545741, -346.5239443744176810 ) ) ;
#76263=CARTESIAN_POINT ( 'NONE',  ( -98.09998604057219040, -296.3788532233318733, -223.3017163505457177 ) ) ;
#76264=CARTESIAN_POINT ( 'NONE',  ( -51.49632924560014402, -275.4755077687397034, -343.0083511409750940 ) ) ;
#76265=CARTESIAN_POINT ( 'NONE',  ( -82.13526567517490662, -277.5161543465504224, -210.8417975660866261 ) ) ;
#76266=CARTESIAN_POINT ( 'NONE',  ( -46.24206423374222652, -275.1418048189901242, -197.5056856308715680 ) ) ;
#76267=CARTESIAN_POINT ( 'NONE',  ( -6.913075853365770129, -275.0593360712501294, -340.2360802745932347 ) ) ;
#76270=CARTESIAN_POINT ( 'NONE',  ( -71.96331869518968460, -274.2334037994623941, -205.9212037993105184 ) ) ;
#76272=CARTESIAN_POINT ( 'NONE',  ( 18.39041245825583815, -286.2768332729150416, -321.0985561820101566 ) ) ;
#76273=CARTESIAN_POINT ( 'NONE',  ( -5.306140316738417795, -274.3191742623328082, -204.7521496480252665 ) ) ;
#76274=CARTESIAN_POINT ( 'NONE',  ( 35.94775315317257025, -287.8491195265457350, -293.9758599403900803 ) ) ;
#76275=CARTESIAN_POINT ( 'NONE',  ( -91.58664357536616762, -289.4656767271319495, -325.0550633259551319 ) ) ;
#76276=CARTESIAN_POINT ( 'NONE',  ( -36.24039811181739168, -300.0457602125951553, -195.0055400566417632 ) ) ;
#76277=CARTESIAN_POINT ( 'NONE',  ( -111.5509562621303274, -294.6811226260339822, -260.3262643196953832 ) ) ;
#76278=CARTESIAN_POINT ( 'NONE',  ( 38.09810183088004720, -280.5664172417576196, -255.7667662894656075 ) ) ;
#76280=CARTESIAN_POINT ( 'NONE',  ( -18.32587242272214212, -278.2968769681713184, -197.7587295238090519 ) ) ;
#76282=CARTESIAN_POINT ( 'NONE',  ( -76.09132718529086503, -288.3774965233114926, -332.6956742695442131 ) ) ;
#76285=CARTESIAN_POINT ( 'NONE',  ( -111.9602290560184770, -288.6489923944097882, -262.8062660380241482 ) ) ;
#76286=CARTESIAN_POINT ( 'NONE',  ( 0.9564155159336718004, -276.0934487225012504, -207.4011140887274678 ) ) ;
#76287=CARTESIAN_POINT ( 'NONE',  ( -0.6423713710800299515, -283.9997005014303681, -337.3965796941538429 ) ) ;
#76288=CARTESIAN_POINT ( 'NONE',  ( -34.10905316332367221, -296.1125408323349006, -195.0069938773381466 ) ) ;
#76289=CARTESIAN_POINT ( 'NONE',  ( -80.62613582809001400, -283.6574293504984894, -329.2071500834630911 ) ) ;
#76290=CARTESIAN_POINT ( 'NONE',  ( -43.54978340593097386, -275.3976124971742365, -196.9830950715867175 ) ) ;
#76291=CARTESIAN_POINT ( 'NONE',  ( -0.4737124017632046158, -275.3585233762697158, -207.1535120387808320 ) ) ;
#76292=CARTESIAN_POINT ( 'NONE',  ( 24.65590105461573245, -286.2147374318741413, -313.6436417353257298 ) ) ;
#76293=CARTESIAN_POINT ( 'NONE',  ( 34.56857836002976114, -283.8288064457119049, -291.8452136433186297 ) ) ;
#76294=CARTESIAN_POINT ( 'NONE',  ( 94.95646885087283806, -298.8069592322501649, -197.1477396936165860 ) ) ;
#76296=CARTESIAN_POINT ( 'NONE',  ( 204.5638081195592122, 295.1839629088547099, -54.00000000004283862 ) ) ;
#76297=CARTESIAN_POINT ( 'NONE',  ( -27.74993937775823127, -294.7670012271443056, -346.8146598934874305 ) ) ;
#76298=CARTESIAN_POINT ( 'NONE',  ( -106.7338867245362479, -286.1705578667221630, -298.0075384234560829 ) ) ;
#76299=CARTESIAN_POINT ( 'NONE',  ( -117.3417001280813423, -270.0523547857346784, -270.3292895737509980 ) ) ;
#76300=CARTESIAN_POINT ( 'NONE',  ( -112.3290637397061573, -277.5392181542181902, -287.1257867821586842 ) ) ;
#76301=EDGE_CURVE ( 'NONE', #37641, #55239, #48370, .T. ) ;
#76302=CARTESIAN_POINT ( 'NONE',  ( -111.2139367995613952, -289.1889487258644067, -251.6181641222729013 ) ) ;
#76303=CARTESIAN_POINT ( 'NONE',  ( -10.70728668976124887, -284.2186311998029851, -339.1270456137751239 ) ) ;
#76304=CARTESIAN_POINT ( 'NONE',  ( -56.84591985023792660, -279.0671290778715274, -341.8115344093550334 ) ) ;
#76305=CARTESIAN_POINT ( 'NONE',  ( -63.02063161816173675, -287.1494456575954359, -198.3944675826213029 ) ) ;
#76306=CARTESIAN_POINT ( 'NONE',  ( -54.98739407203545682, -281.8255670572203826, -197.4128350223410848 ) ) ;
#76307=CARTESIAN_POINT ( 'NONE',  ( -5.116197397439956163, -274.6314201264449935, -200.4288866561637121 ) ) ;
#76308=CARTESIAN_POINT ( 'NONE',  ( -110.6673202174979735, -278.0880351509414936, -294.0350054765586378 ) ) ;
#76309=CARTESIAN_POINT ( 'NONE',  ( -67.86371400210332183, -297.3760549497756642, -338.2700171700143983 ) ) ;
#76310=TOROIDAL_SURFACE ( 'NONE', #35509, 5.343514653206205445, 1.000000000000000000 ) ;
#76313=CARTESIAN_POINT ( 'NONE',  ( -88.75247875321427671, -295.4795912069792507, -214.6372420201819295 ) ) ;
#76314=CARTESIAN_POINT ( 'NONE',  ( 5.427738460538985343, -275.9635083976758665, -329.6584063297124771 ) ) ;
#76315=CARTESIAN_POINT ( 'NONE',  ( -108.8017662732843434, -274.1102221589346755, -242.6203269128297393 ) ) ;
#76316=CARTESIAN_POINT ( 'NONE',  ( 22.80210275257455876, -288.7165801202618809, -227.1389479497133550 ) ) ;
#76317=CARTESIAN_POINT ( 'NONE',  ( -37.66642236224352303, -296.5762281189958571, -346.6800571558220554 ) ) ;
#76318=CARTESIAN_POINT ( 'NONE',  ( -111.9156952345667833, -297.5363409015791376, -287.9314576665448158 ) ) ;
#76319=CARTESIAN_POINT ( 'NONE',  ( -89.21944715022024752, -293.3208142715086524, -216.3568575459673866 ) ) ;
#76320=CARTESIAN_POINT ( 'NONE',  ( 12.54651379812971967, -278.7492407441729938, -214.5830350544112832 ) ) ;
#76321=CARTESIAN_POINT ( 'NONE',  ( -108.6127496141198918, -280.7512964059710043, -248.8727093911112718 ) ) ;
#76322=CARTESIAN_POINT ( 'NONE',  ( -36.43754930487137500, -296.1434028850160303, -195.9214085030576200 ) ) ;
#76323=CARTESIAN_POINT ( 'NONE',  ( -76.10523290413317454, -285.4242658231326004, -335.5195081237679915 ) ) ;
#76325=CARTESIAN_POINT ( 'NONE',  ( 33.99873784092385165, -286.6941633905929052, -287.2361879103874571 ) ) ;
#76326=CARTESIAN_POINT ( 'NONE',  ( -11.30266990606949484, -92.55646609309191319, -359.6964084294213535 ) ) ;
#76328=CARTESIAN_POINT ( 'NONE',  ( 0.1831703079714151194, -286.2330785186373419, -207.6605550212403557 ) ) ;
#76330=CARTESIAN_POINT ( 'NONE',  ( -88.10658806933011533, -284.8224532882052813, -327.9160872133641647 ) ) ;
#76331=CARTESIAN_POINT ( 'NONE',  ( -109.6043162646397207, -273.0284359234773319, -259.5177243449915636 ) ) ;
#76332=CARTESIAN_POINT ( 'NONE',  ( -32.31705935647455163, -284.9090872642121326, -193.9100598209185478 ) ) ;
#76333=CARTESIAN_POINT ( 'NONE',  ( 39.17621167823674000, -282.4162451864140166, -264.2105582314514436 ) ) ;
#76335=CARTESIAN_POINT ( 'NONE',  ( -45.22120558338460938, -281.4743272175518882, -194.4098485349325642 ) ) ;
#76336=CARTESIAN_POINT ( 'NONE',  ( 1.359669952900150802, -280.8873203759857802, -203.7576009053198618 ) ) ;
#76337=CARTESIAN_POINT ( 'NONE',  ( -21.39648532958014826, -286.3380690714489560, -340.3683826091709079 ) ) ;
#76338=CARTESIAN_POINT ( 'NONE',  ( 103.6515131172030095, 116.2435397068051088, -283.0600850077821633 ) ) ;
#76340=CARTESIAN_POINT ( 'NONE',  ( -38.12651595029868190, -276.0424522960996683, -195.5318957835380900 ) ) ;
#76341=CARTESIAN_POINT ( 'NONE',  ( -90.58576820265814433, -230.1752324110255472, -347.6622623265371885 ) ) ;
#76342=CARTESIAN_POINT ( 'NONE',  ( 25.07136067719763872, -279.0160458490407791, -229.3233031774037158 ) ) ;
#76343=CARTESIAN_POINT ( 'NONE',  ( 21.41130435408585697, -294.6565257008296044, -222.1733759581961465 ) ) ;
#76344=CARTESIAN_POINT ( 'NONE',  ( -104.0330092696299715, -295.4965785094855164, -300.4208520403024067 ) ) ;
#76345=CARTESIAN_POINT ( 'NONE',  ( -111.9333636849018205, -290.2965507470121338, -251.4504278974752367 ) ) ;
#76347=CARTESIAN_POINT ( 'NONE',  ( -104.7253641013063543, -295.5973557171842003, -234.2204901812115736 ) ) ;
#76348=CARTESIAN_POINT ( 'NONE',  ( 36.35281526907292005, -285.8892989160941056, -265.5546851710813598 ) ) ;
#76349=CARTESIAN_POINT ( 'NONE',  ( 6.816391997564002381, -296.3050230892768013, -330.0987091538603408 ) ) ;
#76350=CARTESIAN_POINT ( 'NONE',  ( 33.14768931099136040, -285.9631147065874757, -249.5203077237698608 ) ) ;
#76351=CARTESIAN_POINT ( 'NONE',  ( -81.79005048671535860, -286.7472863968405932, -211.8325982079589380 ) ) ;
#76353=CARTESIAN_POINT ( 'NONE',  ( 36.87217313967585852, -294.7398331294729701, -289.9856237895505160 ) ) ;
#76354=CARTESIAN_POINT ( 'NONE',  ( -3.587381373274681096, -283.0864185947573333, -335.1720057463320472 ) ) ;
#76355=CARTESIAN_POINT ( 'NONE',  ( -109.0711666125227310, -295.0035299454532378, -297.3975126226923749 ) ) ;
#76356=CARTESIAN_POINT ( 'NONE',  ( -104.4738742647615624, -291.8406114335153347, -232.9789027493299614 ) ) ;
#76357=CARTESIAN_POINT ( 'NONE',  ( -42.05645968822665992, -292.4865624559037656, -193.5672513942529633 ) ) ;
#76358=CARTESIAN_POINT ( 'NONE',  ( -15.84962372812422515, -288.9330830353967485, -340.1784809887006986 ) ) ;
#76361=CARTESIAN_POINT ( 'NONE',  ( -95.54703591679596286, -297.7492986057359872, -318.8832864868103911 ) ) ;
#76362=CARTESIAN_POINT ( 'NONE',  ( -71.21334725666983445, -272.4098462454447827, -201.6536202754759586 ) ) ;
#76363=CARTESIAN_POINT ( 'NONE',  ( -30.22763583838307966, -279.2029606267645363, -197.4216538472745128 ) ) ;
#76364=EDGE_CURVE ( 'NONE', #85520, #89916, #12090, .T. ) ;
#76365=CARTESIAN_POINT ( 'NONE',  ( 31.19832021748437256, -274.6092782823770904, -235.4069692432904617 ) ) ;
#76366=CARTESIAN_POINT ( 'NONE',  ( -108.8429906471895237, -295.2658498109277616, -252.4692990984672178 ) ) ;
#76367=CARTESIAN_POINT ( 'NONE',  ( -96.23879224412233668, -279.7873534551964099, -315.5495902241452768 ) ) ;
#76368=CARTESIAN_POINT ( 'NONE',  ( -29.84191081088734165, -272.2876770118209606, -196.5057279291170005 ) ) ;
#76369=CARTESIAN_POINT ( 'NONE',  ( -0.5456646725608630399, -295.7569151606389823, -333.9264713786313905 ) ) ;
#76370=CARTESIAN_POINT ( 'NONE',  ( -104.0053867017158780, -298.0428562477958394, -239.7400475757917775 ) ) ;
#76372=CARTESIAN_POINT ( 'NONE',  ( -109.5807499514425132, -297.8437234547807293, -294.6090064566498086 ) ) ;
#76373=CARTESIAN_POINT ( 'NONE',  ( -36.19303743876654522, -296.0663432834716104, -195.1948331483942525 ) ) ;
#76374=CARTESIAN_POINT ( 'NONE',  ( 27.25202138763718551, -294.6704687749886489, -304.6971313117701925 ) ) ;
#76375=CARTESIAN_POINT ( 'NONE',  ( -91.17797276996677169, -289.8427043991016490, -220.1724744300341285 ) ) ;
#76377=CARTESIAN_POINT ( 'NONE',  ( 36.00586127399329683, -276.3367125618950126, -293.5917473238491198 ) ) ;
#76378=CARTESIAN_POINT ( 'NONE',  ( -97.84438154634071338, -273.2876506464223212, -229.4245687950308934 ) ) ;
#76379=CARTESIAN_POINT ( 'NONE',  ( 35.95453964602150876, -283.7562678607716862, -287.9110375050311745 ) ) ;
#76380=CARTESIAN_POINT ( 'NONE',  ( 11.16690718817122452, -281.0815913538260133, -329.5922613597094823 ) ) ;
#76381=CARTESIAN_POINT ( 'NONE',  ( -65.06607605476824574, -276.7534824689196284, -342.1436997471198538 ) ) ;
#76383=CARTESIAN_POINT ( 'NONE',  ( -107.1429753769598534, -283.4594581442398180, -292.2787752632311253 ) ) ;
#76385=CARTESIAN_POINT ( 'NONE',  ( 34.71374241495128388, -279.8291311979189686, -291.9418742854047082 ) ) ;
#76388=CARTESIAN_POINT ( 'NONE',  ( 34.41232581654214329, -273.9124918188405786, -253.9727021139765952 ) ) ;
#76389=CARTESIAN_POINT ( 'NONE',  ( -69.83462975212601975, -279.4801687198992113, -337.9710042952777940 ) ) ;
#76392=CARTESIAN_POINT ( 'NONE',  ( -112.2777488463876097, -271.1302532820440661, -256.2584822934489921 ) ) ;
#76394=CARTESIAN_POINT ( 'NONE',  ( -56.43319225364551528, -279.2976468172718683, -343.1165968422513970 ) ) ;
#76396=CARTESIAN_POINT ( 'NONE',  ( -101.3125932882769860, -287.0088790233717759, -230.1486942156624309 ) ) ;
#76399=CARTESIAN_POINT ( 'NONE',  ( 1.411003838963230450, -286.5346415187040634, -334.6332205906015247 ) ) ;
#76400=VECTOR ( 'NONE', #4696, 1000.000000000000000 ) ;
#76402=CARTESIAN_POINT ( 'NONE',  ( -104.3051457716638595, -294.9430050771975971, -300.5358294888583828 ) ) ;
#76403=CARTESIAN_POINT ( 'NONE',  ( -18.17709084290268962, -286.9422461581812058, -342.1333677983686812 ) ) ;
#76405=CARTESIAN_POINT ( 'NONE',  ( -110.4202099340763965, -294.7685807957072939, -253.4930398996894780 ) ) ;
#76406=CARTESIAN_POINT ( 'NONE',  ( -95.27734773123958689, -283.7089301923844005, -220.6213565429787025 ) ) ;
#76407=CARTESIAN_POINT ( 'NONE',  ( 17.64542445061449882, -282.4556523320346741, -221.1385972562944744 ) ) ;
#76408=CARTESIAN_POINT ( 'NONE',  ( -34.53908727042879434, -281.2572425680131118, -346.2960860593905181 ) ) ;
#76409=CARTESIAN_POINT ( 'NONE',  ( -75.86873968945332081, -289.5823779850818482, -332.3664985767994153 ) ) ;
#76410=CARTESIAN_POINT ( 'NONE',  ( -107.7964547180532264, -280.2564945246516572, -249.1125304233597433 ) ) ;
#76411=CARTESIAN_POINT ( 'NONE',  ( -35.66933598710514275, -280.8764673557497531, -197.2063269233823632 ) ) ;
#76412=CARTESIAN_POINT ( 'NONE',  ( 37.05530737712214773, -289.6891870490071597, -282.6578220402601573 ) ) ;
#76414=CARTESIAN_POINT ( 'NONE',  ( -95.08647638581383887, -273.2418569663221319, -219.4244826898316774 ) ) ;
#76415=CARTESIAN_POINT ( 'NONE',  ( -97.87809587863021932, -291.9347183658455265, -314.0325227466998399 ) ) ;
#76417=CARTESIAN_POINT ( 'NONE',  ( -72.02372285203398405, -291.9805209788416391, -342.4524372437778652 ) ) ;
#76419=CARTESIAN_POINT ( 'NONE',  ( 4.821355287580785465, -274.4838739899860798, -332.5889669121688712 ) ) ;
#76421=CARTESIAN_POINT ( 'NONE',  ( -44.73846493661697821, -293.5440239110451444, -346.2541200324676538 ) ) ;
#76422=CARTESIAN_POINT ( 'NONE',  ( -94.49554268541129431, -296.7020004505471320, -224.8481887995275486 ) ) ;
#76423=CARTESIAN_POINT ( 'NONE',  ( -13.04115754993245524, -290.2507078279832626, -339.9326019558486109 ) ) ;
#76424=CARTESIAN_POINT ( 'NONE',  ( -56.56073321752538163, -285.0634416755692087, -341.8356083843844999 ) ) ;
#76425=CARTESIAN_POINT ( 'NONE',  ( -94.28441374687812981, -292.6738594858829856, -219.4088495424886958 ) ) ;
#76426=CARTESIAN_POINT ( 'NONE',  ( -34.99244343458124717, -293.3962140497518476, -193.8772780442982366 ) ) ;
#76427=CARTESIAN_POINT ( 'NONE',  ( -66.56212616720715403, -291.4917541943732431, -203.4644311691167786 ) ) ;
#76428=CARTESIAN_POINT ( 'NONE',  ( -38.68560912950633224, -288.0354893388805522, -195.3603318999358294 ) ) ;
#76429=CARTESIAN_POINT ( 'NONE',  ( -72.50870513971767650, -279.7663670681044437, -201.8462346356486705 ) ) ;
#76430=CARTESIAN_POINT ( 'NONE',  ( -83.32854787231035232, -293.7561426886059053, -330.3814523584369454 ) ) ;
#76431=CARTESIAN_POINT ( 'NONE',  ( 15.75199781910635899, -282.1583273761293640, -326.1290231143227061 ) ) ;
#76432=CARTESIAN_POINT ( 'NONE',  ( 23.27598800998567796, -276.8240812207150157, -227.4863352907541412 ) ) ;
#76433=CARTESIAN_POINT ( 'NONE',  ( -105.5937364680635966, -275.2662352645559167, -254.8156830097664738 ) ) ;
#76434=CARTESIAN_POINT ( 'NONE',  ( -64.67198163286256829, -275.5446747933210645, -341.0802284867209551 ) ) ;
#76436=CARTESIAN_POINT ( 'NONE',  ( 3.419358850103377367, -281.9956956474497360, -331.0566624037581960 ) ) ;
#76437=CARTESIAN_POINT ( 'NONE',  ( -112.4014579835181138, -279.5640888472843812, -285.7242941006983870 ) ) ;
#76438=CARTESIAN_POINT ( 'NONE',  ( -107.7056409591531434, -284.0048322855715810, -239.5405368461725288 ) ) ;
#76439=CARTESIAN_POINT ( 'NONE',  ( -64.46352547408663725, -293.4533958526740776, -201.4824504845877016 ) ) ;
#76440=CARTESIAN_POINT ( 'NONE',  ( 25.47342839486007549, -276.5767241440461248, -227.2021668403941135 ) ) ;
#76441=CARTESIAN_POINT ( 'NONE',  ( 6.935854778539218835, -275.9557569601988689, -207.9038340390339386 ) ) ;
#76442=CARTESIAN_POINT ( 'NONE',  ( -9.990333026611466494, -276.5181379909447514, -338.0570498900360121 ) ) ;
#76443=CARTESIAN_POINT ( 'NONE',  ( -104.1810135834413984, -298.9992136855112221, -236.5925114287485087 ) ) ;
#76444=CARTESIAN_POINT ( 'NONE',  ( -102.5773445585654713, -283.0426510456817937, -233.5897554845238346 ) ) ;
#76445=CARTESIAN_POINT ( 'NONE',  ( 20.36565442307731288, -292.5286107965130213, -219.3941163929616209 ) ) ;
#76446=CARTESIAN_POINT ( 'NONE',  ( 38.55250176099807646, -289.2384661410605986, -277.1809811570702777 ) ) ;
#76447=CARTESIAN_POINT ( 'NONE',  ( 35.21563908366541540, -292.3349182322745037, -259.8893177433520236 ) ) ;
#76449=CARTESIAN_POINT ( 'NONE',  ( -27.90373146379274871, -290.7443363928971394, -194.4821909894145335 ) ) ;
#76450=CARTESIAN_POINT ( 'NONE',  ( 22.60771860761217056, -292.6376985038773455, -228.6479026957655094 ) ) ;
#76452=CARTESIAN_POINT ( 'NONE',  ( -34.66379058456840312, -290.0989053819855599, -347.0052391598403574 ) ) ;
#76453=CARTESIAN_POINT ( 'NONE',  ( -109.9245484245452786, -278.7741910939839158, -278.7964727294116756 ) ) ;
#76455=CARTESIAN_POINT ( 'NONE',  ( -108.0952018556565690, -295.0930993413451802, -300.0863635499195539 ) ) ;
#76456=CARTESIAN_POINT ( 'NONE',  ( -95.74458746593975889, -285.8801130297811142, -220.2570947718829473 ) ) ;
#76457=CARTESIAN_POINT ( 'NONE',  ( 37.80523059895784144, -288.0950207990633771, -287.1151143867770656 ) ) ;
#76458=CARTESIAN_POINT ( 'NONE',  ( -70.22064498324230897, -283.8310730745346291, -335.5752726161098280 ) ) ;
#76459=CARTESIAN_POINT ( 'NONE',  ( 202.0776253717283737, 293.7063013533117442, -83.21832582370875286 ) ) ;
#76460=CARTESIAN_POINT ( 'NONE',  ( -57.39736010472714156, -168.6502712723204240, -363.1223024648248838 ) ) ;
#76461=CARTESIAN_POINT ( 'NONE',  ( -70.73824396572096873, -195.6031298962179790, -356.6742706091125683 ) ) ;
#76462=CARTESIAN_POINT ( 'NONE',  ( 22.59225271492110210, -275.3342239518406132, -312.4066643714056681 ) ) ;
#76463=CARTESIAN_POINT ( 'NONE',  ( 29.43017786110765499, -274.8786252294602832, -300.6223536225385828 ) ) ;
#76464=CARTESIAN_POINT ( 'NONE',  ( -89.56193029040233000, -296.8474396712807106, -213.7860823365475653 ) ) ;
#76465=CARTESIAN_POINT ( 'NONE',  ( 66.02812564630266934, 45.92910118373598749, -315.8466591048211285 ) ) ;
#76466=CARTESIAN_POINT ( 'NONE',  ( 36.81141119533734951, -273.9998289900178747, -251.5299110285778568 ) ) ;
#76467=CARTESIAN_POINT ( 'NONE',  ( -111.3550334602798699, -274.3120101394163157, -270.3834770935375218 ) ) ;
#76469=CARTESIAN_POINT ( 'NONE',  ( -103.9678297180685149, -274.1282815347021256, -232.2748936603652226 ) ) ;
#76471=CARTESIAN_POINT ( 'NONE',  ( 23.56425921944132540, -288.6042495599207882, -310.7380619729346449 ) ) ;
#76472=CARTESIAN_POINT ( 'NONE',  ( -65.53471439865862180, -296.2143623095975045, -341.8547662142683521 ) ) ;
#76473=CARTESIAN_POINT ( 'NONE',  ( -65.52530806583628475, -298.1858490065776550, -198.7135921590706289 ) ) ;
#76474=CARTESIAN_POINT ( 'NONE',  ( -10.48802672819066828, -294.8584447510136215, -338.2424867772592165 ) ) ;
#76476=CARTESIAN_POINT ( 'NONE',  ( 18.94648717451537223, -276.7748672446655860, -219.8763795095855755 ) ) ;
#76478=CARTESIAN_POINT ( 'NONE',  ( -53.74124167373921068, -279.3549166971457680, -195.1362407033382453 ) ) ;
#76479=CARTESIAN_POINT ( 'NONE',  ( -72.94594343254587443, -278.4774928210591725, -334.3735629527138826 ) ) ;
#76480=CARTESIAN_POINT ( 'NONE',  ( -20.33085777978403996, -278.5968313288817058, -344.4732414441789956 ) ) ;
#76481=CARTESIAN_POINT ( 'NONE',  ( -90.19379001330752033, -275.8146220283531989, -324.1470010600972955 ) ) ;
#76482=CARTESIAN_POINT ( 'NONE',  ( -93.82995333313432695, -273.7005150137832743, -224.0051138216794868 ) ) ;
#76483=CARTESIAN_POINT ( 'NONE',  ( -97.35281674859676571, -295.7168740479199869, -227.7695601353353538 ) ) ;
#76485=CARTESIAN_POINT ( 'NONE',  ( -94.45170733341134905, -278.0764875778563692, -315.8502725316577084 ) ) ;
#76486=CARTESIAN_POINT ( 'NONE',  ( -38.92685501898818501, -287.7564819854090956, -346.8515458700260865 ) ) ;
#76487=CARTESIAN_POINT ( 'NONE',  ( -16.36188926982008596, -276.3233417246316890, -198.3013326868602064 ) ) ;
#76489=CARTESIAN_POINT ( 'NONE',  ( -88.78185020040575637, -288.9945901950816278, -322.3852728273838011 ) ) ;
#76490=CARTESIAN_POINT ( 'NONE',  ( -95.26342772700883188, -283.2157722314795478, -320.9416108504484555 ) ) ;
#76491=CARTESIAN_POINT ( 'NONE',  ( 1.615889759993562658, -280.7638497990469091, -333.3517107786541374 ) ) ;
#76492=CARTESIAN_POINT ( 'NONE',  ( 25.64998266121680714, -279.6062374946538398, -232.2173182046038278 ) ) ;
#76493=CARTESIAN_POINT ( 'NONE',  ( -63.03743404493653202, -283.7949028775299212, -200.4416891151780931 ) ) ;
#76494=CARTESIAN_POINT ( 'NONE',  ( -63.17603437508145703, -287.7159632494962125, -199.8964818378199766 ) ) ;
#76495=CARTESIAN_POINT ( 'NONE',  ( -81.53915246214216950, -280.6408812515650197, -211.6993741935708044 ) ) ;
#76496=CARTESIAN_POINT ( 'NONE',  ( 14.04872217819529112, -294.7731795276428102, -215.6636020820816952 ) ) ;
#76497=CARTESIAN_POINT ( 'NONE',  ( -47.95478125794594604, -278.1589320212169696, -195.0661304319107785 ) ) ;
#76498=CARTESIAN_POINT ( 'NONE',  ( 22.55411767426107517, -276.7882349552257324, -312.3572672008701829 ) ) ;
#76499=CARTESIAN_POINT ( 'NONE',  ( -52.52185957043352715, -285.2461834177107107, -344.0321814315896063 ) ) ;
#76501=CARTESIAN_POINT ( 'NONE',  ( -102.5432373721015864, -291.9646349741823883, -308.6492832714856718 ) ) ;
#76502=CARTESIAN_POINT ( 'NONE',  ( -111.4864994332881167, -294.7012415681579682, -258.7371390073324164 ) ) ;
#76504=CARTESIAN_POINT ( 'NONE',  ( 39.18570460005456368, -286.8358922961920712, -277.2687330363582987 ) ) ;
#76505=CARTESIAN_POINT ( 'NONE',  ( -82.19932917432734598, -289.8288252163771404, -211.6941314157282363 ) ) ;
#76507=CARTESIAN_POINT ( 'NONE',  ( 14.06438449782166522, -274.9971618522870358, -322.9549043105789110 ) ) ;
#76508=CARTESIAN_POINT ( 'NONE',  ( 28.23833922142655695, -292.1590438555282390, -305.2577342872530721 ) ) ;
#76511=CARTESIAN_POINT ( 'NONE',  ( -33.55424171836384062, -290.5788983845924349, -194.1485014912937856 ) ) ;
#76512=CARTESIAN_POINT ( 'NONE',  ( -52.27045588907994045, -287.4579419282569006, -198.0868302691719123 ) ) ;
#76513=CARTESIAN_POINT ( 'NONE',  ( -36.12583683735016393, -287.2770035012818539, -346.3509979411987274 ) ) ;
#76514=CARTESIAN_POINT ( 'NONE',  ( -97.06356115614984503, -286.5740936262721448, -227.3434023554003147 ) ) ;
#76516=CARTESIAN_POINT ( 'NONE',  ( -30.52640065874925668, -286.9432289559196647, -197.4668589413124380 ) ) ;
#76517=CARTESIAN_POINT ( 'NONE',  ( 38.06566468328554720, -295.5310859627203968, -270.2858865059675395 ) ) ;
#76518=CARTESIAN_POINT ( 'NONE',  ( -95.95319992546896515, -275.9797408285566576, -318.0679287200999852 ) ) ;
#76519=CARTESIAN_POINT ( 'NONE',  ( 37.88592085992544867, -276.0904415627179560, -286.7490583984293266 ) ) ;
#76520=CARTESIAN_POINT ( 'NONE',  ( -47.52466074643158578, -290.0036669445614166, -195.4376326333212717 ) ) ;
#76521=CARTESIAN_POINT ( 'NONE',  ( -106.1755779162270699, -278.9973941920438847, -235.7329874477496503 ) ) ;
#76522=CARTESIAN_POINT ( 'NONE',  ( -95.20184817669124300, -297.8789533473575943, -317.5410344465990420 ) ) ;
#76525=CARTESIAN_POINT ( 'NONE',  ( -46.77166153146829686, -284.6148853284377083, -197.4243411303504558 ) ) ;
#76526=CARTESIAN_POINT ( 'NONE',  ( -109.0189822456722055, -276.4407982536561690, -289.6803496066063985 ) ) ;
#76527=CARTESIAN_POINT ( 'NONE',  ( 3.436350252227038382, -280.5041807352507135, -333.3681085133127340 ) ) ;
#76529=CARTESIAN_POINT ( 'NONE',  ( -15.95297372255607904, -272.8036259670304275, -197.0585413385411471 ) ) ;
#76531=CARTESIAN_POINT ( 'NONE',  ( 36.11709217213325473, -295.1490506209334512, -276.2359443631333988 ) ) ;
#76532=CARTESIAN_POINT ( 'NONE',  ( 38.11894000997226328, -280.6451961972731510, -284.1155205264357164 ) ) ;
#76533=CARTESIAN_POINT ( 'NONE',  ( -35.63314603846480111, -295.9714821568629191, -343.5890166210859888 ) ) ;
#76534=CARTESIAN_POINT ( 'NONE',  ( -112.1195825992270727, -297.6637503386282333, -286.5341377351184633 ) ) ;
#76535=CARTESIAN_POINT ( 'NONE',  ( 8.930710037563439840, -298.4806182316301602, -197.3624746187491610 ) ) ;
#76536=CARTESIAN_POINT ( 'NONE',  ( -94.08592463948411933, -293.2324258640568360, -221.3193639787115217 ) ) ;
#76537=CARTESIAN_POINT ( 'NONE',  ( -12.70571787137886233, -286.5304776923700274, -197.4086102618328482 ) ) ;
#76538=CARTESIAN_POINT ( 'NONE',  ( 37.01121162820782473, -273.5066983485751280, -255.8026154350708339 ) ) ;
#76539=CARTESIAN_POINT ( 'NONE',  ( 0.7174463734385814195, -288.3928920754133856, -337.3579173016635764 ) ) ;
#76540=CARTESIAN_POINT ( 'NONE',  ( 35.91606645810338705, -286.5840264297027602, -268.3178157173430236 ) ) ;
#76541=CARTESIAN_POINT ( 'NONE',  ( -73.68679976405829279, -289.5694842327730498, -204.7559780725573830 ) ) ;
#76543=CARTESIAN_POINT ( 'NONE',  ( -108.4555765497910471, -262.4588243622614527, -317.8183916042563055 ) ) ;
#76544=CARTESIAN_POINT ( 'NONE',  ( -42.67465990898582362, -288.6287547114201857, -343.2784098232261272 ) ) ;
#76546=CARTESIAN_POINT ( 'NONE',  ( -109.7592728075075712, -285.8156345934768297, -244.8951528555565176 ) ) ;
#76547=CARTESIAN_POINT ( 'NONE',  ( 1.591137889000544980, -291.6176674398516298, -204.1410555231681769 ) ) ;
#76548=CARTESIAN_POINT ( 'NONE',  ( 8.053437036477692601, -282.2609072772607988, -209.0932365007826661 ) ) ;
#76549=CARTESIAN_POINT ( 'NONE',  ( 36.84891077491612066, -282.6320521936957562, -251.6781972200875543 ) ) ;
#76550=CARTESIAN_POINT ( 'NONE',  ( -34.84866714145898214, -282.8533203320646976, -343.3309722403500359 ) ) ;
#76551=CARTESIAN_POINT ( 'NONE',  ( 18.76524934551564883, -276.8593582428042055, -220.5146185197979776 ) ) ;
#76552=CARTESIAN_POINT ( 'NONE',  ( -101.6282676053475029, -295.9937785143127371, -312.8395856388088987 ) ) ;
#76553=CARTESIAN_POINT ( 'NONE',  ( -106.2110834230515479, -288.9515250770970738, -241.4368797290185569 ) ) ;
#76554=CARTESIAN_POINT ( 'NONE',  ( -87.59404735942686671, -272.1269183271066368, -216.7954519976267989 ) ) ;
#76556=EDGE_LOOP ( 'NONE', ( #33784, #49183 ) ) ;
#76558=CARTESIAN_POINT ( 'NONE',  ( -105.9337740114443989, -286.8545154619316691, -241.3072221966463360 ) ) ;
#76559=CARTESIAN_POINT ( 'NONE',  ( 34.16824444149040829, -294.9842794391035454, -298.0706891945355892 ) ) ;
#76560=CARTESIAN_POINT ( 'NONE',  ( -64.08495003180270544, -284.0618858529895192, -338.3956037442119964 ) ) ;
#76561=CARTESIAN_POINT ( 'NONE',  ( 33.96123670155220964, -274.9744102214193617, -298.9422266537117139 ) ) ;
#76562=CARTESIAN_POINT ( 'NONE',  ( -95.58914123365204318, -291.8825688328802244, -220.1359251740089462 ) ) ;
#76563=CARTESIAN_POINT ( 'NONE',  ( -51.91215501165626023, -284.0073354190644750, -195.9570332820456429 ) ) ;
#76564=CARTESIAN_POINT ( 'NONE',  ( -84.25682486062854082, -291.7602647917484546, -209.2634871296109509 ) ) ;
#76565=CARTESIAN_POINT ( 'NONE',  ( -108.4490344042040846, -291.1051805550153517, -253.6983097913259542 ) ) ;
#76567=FACE_OUTER_BOUND ( 'NONE', #72404, .T. ) ;
#76568=CARTESIAN_POINT ( 'NONE',  ( 45.77323534221019941, 10.84377598319223779, -328.4943775524195644 ) ) ;
#76569=CARTESIAN_POINT ( 'NONE',  ( -97.48588656273726372, -285.4390590387739053, -317.3226404613002956 ) ) ;
#76570=CARTESIAN_POINT ( 'NONE',  ( -54.49178911615187104, -280.7666405000204009, -345.3538533559490702 ) ) ;
#76572=CARTESIAN_POINT ( 'NONE',  ( 32.52172574600692201, -280.7676859438883525, -292.7373300214495657 ) ) ;
#76573=CARTESIAN_POINT ( 'NONE',  ( -51.31294624711899388, -276.8928262412638901, -346.0615048595248027 ) ) ;
#76574=CARTESIAN_POINT ( 'NONE',  ( -34.26277092075687136, -282.0910846996497980, -195.5782878711285093 ) ) ;
#76575=CARTESIAN_POINT ( 'NONE',  ( 162.7603103009924155, 217.9236943496693186, -203.6326850931731371 ) ) ;
#76576=CARTESIAN_POINT ( 'NONE',  ( 24.12861320391544595, -279.5190817099143601, -224.9738193956834778 ) ) ;
#76577=CARTESIAN_POINT ( 'NONE',  ( -74.34967771691152905, -283.5776698133333866, -205.5214846736406855 ) ) ;
#76578=CARTESIAN_POINT ( 'NONE',  ( -29.21748939662639444, -299.9126702956965573, -194.3720490655677224 ) ) ;
#76579=CARTESIAN_POINT ( 'NONE',  ( -93.12532351689074517, -296.3743056158288027, -317.5628645845365554 ) ) ;
#76581=CARTESIAN_POINT ( 'NONE',  ( -107.0336605112414361, -289.5447476143401673, -247.0314344055476568 ) ) ;
#76582=CARTESIAN_POINT ( 'NONE',  ( 35.10773432549471096, -276.5310751071872346, -296.2939267924919591 ) ) ;
#76583=CARTESIAN_POINT ( 'NONE',  ( 21.48118147675633338, -274.9464567763436094, -227.1307050802612082 ) ) ;
#76584=CARTESIAN_POINT ( 'NONE',  ( 38.42816383699886984, -274.6254615369954877, -282.5439436668503390 ) ) ;
#76586=CARTESIAN_POINT ( 'NONE',  ( -75.79491863347708147, -271.5390859265188510, -205.9094166353348498 ) ) ;
#76590=CARTESIAN_POINT ( 'NONE',  ( 32.53011433091749183, -282.9266804448087669, -292.7111277205769397 ) ) ;
#76591=CARTESIAN_POINT ( 'NONE',  ( 38.17307873055065670, -283.1993127890175970, -261.4462975323013438 ) ) ;
#76592=CARTESIAN_POINT ( 'NONE',  ( -89.73012471310292426, -284.6376622228160045, -219.3047079616582096 ) ) ;
#76593=CARTESIAN_POINT ( 'NONE',  ( 23.10954566211194106, -274.5370568693433029, -312.7818725018061059 ) ) ;
#76594=CARTESIAN_POINT ( 'NONE',  ( -61.92173439816566827, -285.2353665560385139, -340.4629983659432355 ) ) ;
#76595=CARTESIAN_POINT ( 'NONE',  ( -41.91880686746605988, -275.5907144707901466, -343.9248900447914821 ) ) ;
#76597=CARTESIAN_POINT ( 'NONE',  ( -24.55598058415324658, -275.2987054726415863, -198.1237777896839702 ) ) ;
#76599=CARTESIAN_POINT ( 'NONE',  ( -64.69442686515992591, -280.5068941690625479, -198.4998000430934155 ) ) ;
#76602=CARTESIAN_POINT ( 'NONE',  ( -66.73212955454549444, -287.5315903770040791, -200.5291185837035357 ) ) ;
#76603=CARTESIAN_POINT ( 'NONE',  ( -45.11803947041191520, -294.3501712361127716, -343.1587358381387958 ) ) ;
#76604=CARTESIAN_POINT ( 'NONE',  ( -108.2699144452730451, -290.2790998385033845, -240.6541962289265939 ) ) ;
#76605=CARTESIAN_POINT ( 'NONE',  ( 31.93084578902593407, -285.4472717793988181, -244.1531621404348016 ) ) ;
#76606=CARTESIAN_POINT ( 'NONE',  ( -35.90390096878096671, -284.6452615214085426, -196.7859343106696031 ) ) ;
#76607=CARTESIAN_POINT ( 'NONE',  ( -111.2562393032154802, -288.8533123169111150, -265.6490732066125133 ) ) ;
#76608=CARTESIAN_POINT ( 'NONE',  ( -108.4742786379083270, -285.5197404811117963, -288.4521870626683153 ) ) ;
#76609=CARTESIAN_POINT ( 'NONE',  ( -7.397242079258217196, -274.6593686441573254, -339.1378552451679980 ) ) ;
#76611=CARTESIAN_POINT ( 'NONE',  ( 7.094123897701084758, -285.0456621174336647, -208.3937916942269339 ) ) ;
#76612=CARTESIAN_POINT ( 'NONE',  ( -37.62631890171964955, -300.0487446769467397, -195.3616536796459116 ) ) ;
#76613=CARTESIAN_POINT ( 'NONE',  ( 29.79600266233247652, -285.1064498350896201, -236.5593830046665005 ) ) ;
#76614=CARTESIAN_POINT ( 'NONE',  ( -5.466883223478672171, -281.4233898864263779, -204.4262675901926229 ) ) ;
#76615=CARTESIAN_POINT ( 'NONE',  ( -72.29812593220761130, -291.5136513980145310, -336.9193165610674896 ) ) ;
#76618=CARTESIAN_POINT ( 'NONE',  ( -30.69284333728993985, -296.8888606969608190, -345.6280224039527411 ) ) ;
#76619=CARTESIAN_POINT ( 'NONE',  ( -16.33785894445908227, -278.3234877734162183, -198.3622339514360249 ) ) ;
#76620=CARTESIAN_POINT ( 'NONE',  ( 35.30330697479982405, -292.4312454658624461, -245.1627872002271431 ) ) ;
#76621=CARTESIAN_POINT ( 'NONE',  ( -106.5490206060877654, -295.2917880932865273, -244.5859655528838630 ) ) ;
#76622=CARTESIAN_POINT ( 'NONE',  ( 35.05575875174248068, -280.0713080165008364, -257.7178815881530909 ) ) ;
#76623=CARTESIAN_POINT ( 'NONE',  ( -8.388608893812747880, -272.5138707157639715, -201.7274727217701695 ) ) ;
#76624=CARTESIAN_POINT ( 'NONE',  ( 9.147930413843498698, -294.0208891608623389, -213.3744949042412884 ) ) ;
#76625=CARTESIAN_POINT ( 'NONE',  ( -69.85430415644619018, -291.9805209788416391, -337.9475929042657754 ) ) ;
#76626=CARTESIAN_POINT ( 'NONE',  ( -112.5241843097678043, -294.8635703285478940, -283.7101061273240248 ) ) ;
#76627=CARTESIAN_POINT ( 'NONE',  ( 38.43227163499855692, -291.7200093274458368, -264.6796379699028989 ) ) ;
#76628=CARTESIAN_POINT ( 'NONE',  ( -88.35200724408710471, -292.7460186934327453, -217.2499060422842661 ) ) ;
#76630=CARTESIAN_POINT ( 'NONE',  ( -92.68533390788199711, -292.0352914715937231, -222.5104761124463266 ) ) ;
#76631=CARTESIAN_POINT ( 'NONE',  ( -35.95529233870315267, -281.0549909850892618, -345.7164044554401698 ) ) ;
#76632=CARTESIAN_POINT ( 'NONE',  ( -30.80697332525654275, -292.1370550477507777, -197.6541902135197404 ) ) ;
#76633=CARTESIAN_POINT ( 'NONE',  ( 39.41170925864951613, -281.4751448022304885, -264.2036714734219913 ) ) ;
#76634=CARTESIAN_POINT ( 'NONE',  ( -108.2093362901456715, -283.8346291699731410, -300.5561501315042960 ) ) ;
#76635=CARTESIAN_POINT ( 'NONE',  ( -28.99326453416362526, -286.9459128857212136, -344.7273203098748127 ) ) ;
#76636=CARTESIAN_POINT ( 'NONE',  ( 32.54576606641337122, -279.6378196074267066, -239.7269896305699035 ) ) ;
#76637=CARTESIAN_POINT ( 'NONE',  ( 38.78199126036250988, -286.5947429566154483, -280.0976348922514489 ) ) ;
#76639=CARTESIAN_POINT ( 'NONE',  ( 26.92125939201894980, -294.6597212768976419, -233.9702917787960530 ) ) ;
#76640=CARTESIAN_POINT ( 'NONE',  ( -67.45952374629314363, -278.8648203355996884, -340.5859212533017626 ) ) ;
#76641=CARTESIAN_POINT ( 'NONE',  ( -102.1727021121564007, -278.6770270542980938, -236.6500620236490704 ) ) ;
#76642=CARTESIAN_POINT ( 'NONE',  ( 39.65592328351496576, -293.6822302851240352, -267.4344854004200442 ) ) ;
#76643=CARTESIAN_POINT ( 'NONE',  ( 0.1325363614081735142, -280.6372298423601137, -335.9885296395385126 ) ) ;
#76644=CARTESIAN_POINT ( 'NONE',  ( 26.44536948771673934, -292.1187500288311298, -234.2767393968833005 ) ) ;
#76645=CARTESIAN_POINT ( 'NONE',  ( -111.9561552009020744, -294.4544703409337103, -277.9560993184263680 ) ) ;
#76646=ORIENTED_EDGE ( 'NONE', *, *, #90226, .T. ) ;
#76648=CARTESIAN_POINT ( 'NONE',  ( -10.47319891448835705, -294.1995238890440874, -338.3027994766823099 ) ) ;
#76649=FACE_OUTER_BOUND ( 'NONE', #11723, .T. ) ;
#76650=CARTESIAN_POINT ( 'NONE',  ( -21.39648532958014826, -292.3380690714489560, -340.3683826091709079 ) ) ;
#76651=CARTESIAN_POINT ( 'NONE',  ( 53.25449529029830131, -298.2191232718067226, -193.6104392773155496 ) ) ;
#76652=CARTESIAN_POINT ( 'NONE',  ( 27.23953207529913101, -280.2189802970960955, -310.0782911197750877 ) ) ;
#76653=CARTESIAN_POINT ( 'NONE',  ( 28.26696695656664104, -288.3495996160002619, -230.9041700946816604 ) ) ;
#76654=CARTESIAN_POINT ( 'NONE',  ( 33.08134115626550198, -287.6416882212055270, -289.7735396969575277 ) ) ;
#76655=CARTESIAN_POINT ( 'NONE',  ( -108.4845937189351446, -279.8207897370473916, -289.5808069834986895 ) ) ;
#76656=CARTESIAN_POINT ( 'NONE',  ( -81.13979601274394327, -293.6706808318216986, -330.8059159125374435 ) ) ;
#76657=CARTESIAN_POINT ( 'NONE',  ( -88.84679080605808110, -299.0772781492377135, -217.1369353207897177 ) ) ;
#76658=CARTESIAN_POINT ( 'NONE',  ( -110.5656749594325987, -277.2718436589311750, -276.0947032256683542 ) ) ;
#76660=CARTESIAN_POINT ( 'NONE',  ( -105.6079596317261320, -272.8462587157188182, -234.6268191249995141 ) ) ;
#76661=CARTESIAN_POINT ( 'NONE',  ( -81.23730489548655953, -291.5737004659950458, -330.5458750137212292 ) ) ;
#76662=CARTESIAN_POINT ( 'NONE',  ( 37.00790010273387765, -295.3639497309682724, -287.1107183995169976 ) ) ;
#76663=CARTESIAN_POINT ( 'NONE',  ( 202.3291156054731346, 292.0658875081724091, -53.99999999997604760 ) ) ;
#76664=CARTESIAN_POINT ( 'NONE',  ( -109.3786519940150868, -291.3711560438437118, -257.6392874493740237 ) ) ;
#76667=CARTESIAN_POINT ( 'NONE',  ( -80.57457805637038462, -298.1344604248849350, -206.7028221423462924 ) ) ;
#76668=CARTESIAN_POINT ( 'NONE',  ( -109.2509330367413583, -288.9988741009902355, -246.3356692337193294 ) ) ;
#76669=CARTESIAN_POINT ( 'NONE',  ( 53.55226604457176620, -299.4943067948125304, -193.3772322354090250 ) ) ;
#76672=CARTESIAN_POINT ( 'NONE',  ( -9.795398941516131330, -290.2189021077890629, -341.5222663965483321 ) ) ;
#76673=CARTESIAN_POINT ( 'NONE',  ( -119.3990491898856732, -281.0519495502701943, -270.3937649182068412 ) ) ;
#76675=CARTESIAN_POINT ( 'NONE',  ( -111.0020447630474507, -286.7230776743869001, -257.0910900317908272 ) ) ;
#76677=CARTESIAN_POINT ( 'NONE',  ( 23.40413665144833288, -285.5039181236483046, -223.9872091681073414 ) ) ;
#76678=CARTESIAN_POINT ( 'NONE',  ( 10.68060858862410001, -272.7169704728086685, -212.9008518456541026 ) ) ;
#76679=CARTESIAN_POINT ( 'NONE',  ( -70.14716857114906645, -275.5366153623551213, -203.5395986793191412 ) ) ;
#76680=CARTESIAN_POINT ( 'NONE',  ( -111.5604172484394780, -288.5496116041332471, -276.7292282745677312 ) ) ;
#76681=CARTESIAN_POINT ( 'NONE',  ( -74.70608869245306494, -279.4043998861710065, -336.2717237171921170 ) ) ;
#76683=CARTESIAN_POINT ( 'NONE',  ( 9.276538532253212566, -280.7132319616817995, -214.1192516020252583 ) ) ;
#76684=CARTESIAN_POINT ( 'NONE',  ( -11.69963187783426939, -279.7435149230977345, -201.8504652150937204 ) ) ;
#76685=CARTESIAN_POINT ( 'NONE',  ( 23.28217962871956459, -277.2617318547763148, -317.3530255161510922 ) ) ;
#76686=CARTESIAN_POINT ( 'NONE',  ( 24.28150080872926253, -279.7392426791169555, -224.8573837862583389 ) ) ;
#76687=CARTESIAN_POINT ( 'NONE',  ( -40.60242197809582620, -139.1959913163171620, -361.5915507396188104 ) ) ;
#76688=CARTESIAN_POINT ( 'NONE',  ( -3.939357049675801026, -275.4232249478636732, -201.2300602596499743 ) ) ;
#76690=CARTESIAN_POINT ( 'NONE',  ( -80.87090453512651322, -274.9935689934691254, -207.6239886869931013 ) ) ;
#76691=CARTESIAN_POINT ( 'NONE',  ( -20.25526795762937127, -294.7662352645559167, -195.3538533559490702 ) ) ;
#76694=CARTESIAN_POINT ( 'NONE',  ( 21.42950459440442401, -289.2442935791040100, -314.2018988088595393 ) ) ;
#76695=CARTESIAN_POINT ( 'NONE',  ( 26.60432939761541959, -289.8590355010832695, -311.5054610518041613 ) ) ;
#76696=CARTESIAN_POINT ( 'NONE',  ( -102.9405496951424510, -289.4642245306970381, -302.6207460539445719 ) ) ;
#76697=CARTESIAN_POINT ( 'NONE',  ( -64.51958215165524280, -285.2143914695812441, -198.3685651946223061 ) ) ;
#76699=CARTESIAN_POINT ( 'NONE',  ( 27.54889578111157533, -280.4264633211897149, -305.5129454716814621 ) ) ;
#76700=CARTESIAN_POINT ( 'NONE',  ( 32.57050280545230692, -289.7394053802656799, -295.3240777454739145 ) ) ;
#76701=CARTESIAN_POINT ( 'NONE',  ( -3.318327443655574971, -281.0742748396984894, -335.7443440979537286 ) ) ;
#76702=CARTESIAN_POINT ( 'NONE',  ( -110.8449567856905418, -279.8994717789595370, -267.9084008339096954 ) ) ;
#76703=CARTESIAN_POINT ( 'NONE',  ( -70.47510922770024422, -277.9936729455083650, -335.4776722777727400 ) ) ;
#76704=CARTESIAN_POINT ( 'NONE',  ( -107.9949577011233117, -289.7255264533641821, -240.7616938007201099 ) ) ;
#76705=CARTESIAN_POINT ( 'NONE',  ( -113.6604452798630120, -285.4668030306847868, -261.4387887609575500 ) ) ;
#76706=CARTESIAN_POINT ( 'NONE',  ( -71.04493448815912870, -286.1115718872038656, -201.1974071419211043 ) ) ;
#76707=CARTESIAN_POINT ( 'NONE',  ( 32.23196691350072030, -282.0138363489546123, -292.6279110291256416 ) ) ;
#76710=CARTESIAN_POINT ( 'NONE',  ( -102.7203795270322502, -291.9049064666373852, -308.7523481915845878 ) ) ;
#76711=CARTESIAN_POINT ( 'NONE',  ( 1.464502773491773935, -291.2438057354800662, -204.3659269331617168 ) ) ;
#76712=CARTESIAN_POINT ( 'NONE',  ( 28.07682607989820767, -274.1655286602704109, -237.4396223276166893 ) ) ;
#76713=CARTESIAN_POINT ( 'NONE',  ( -86.33675949824396412, -295.0605327958493831, -329.6299710470999003 ) ) ;
#76714=CARTESIAN_POINT ( 'NONE',  ( -79.91562587690184216, -289.9447944676441580, -210.1473665590815756 ) ) ;
#76715=CARTESIAN_POINT ( 'NONE',  ( -17.97665795845529502, -293.0388964498699806, -341.7961874714746955 ) ) ;
#76717=CARTESIAN_POINT ( 'NONE',  ( -74.90600990107076029, -290.7694777610180381, -333.4318354204780235 ) ) ;
#76718=CARTESIAN_POINT ( 'NONE',  ( -37.37352853689063892, -300.5519495502701943, -195.3611179825600175 ) ) ;
#76719=CARTESIAN_POINT ( 'NONE',  ( -54.03111960814487702, -291.2664552906873610, -343.5339230191971751 ) ) ;
#76720=CARTESIAN_POINT ( 'NONE',  ( -28.04984531623601995, -290.1695408249292427, -195.7185740383867767 ) ) ;
#76721=CARTESIAN_POINT ( 'NONE',  ( 28.71352174661529588, -296.0250602192240876, -305.9899822279509181 ) ) ;
#76722=CARTESIAN_POINT ( 'NONE',  ( -11.95161078791422860, -287.3321895460314863, -201.6679464778129045 ) ) ;
#76723=CARTESIAN_POINT ( 'NONE',  ( -44.59279534605742157, -297.1437322773941787, -345.2293602885483779 ) ) ;
#76724=CARTESIAN_POINT ( 'NONE',  ( -43.92474550783400389, -275.9493555785821854, -195.2418423320020509 ) ) ;
#76725=CARTESIAN_POINT ( 'NONE',  ( 16.66434370630601336, -275.0998115301671874, -324.7615546432394353 ) ) ;
#76726=CARTESIAN_POINT ( 'NONE',  ( 76.10082423805694418, -298.6357017837653984, -193.5375264744100434 ) ) ;
#76727=CARTESIAN_POINT ( 'NONE',  ( -13.47961245494971472, -274.9780316423373279, -340.4762083061955309 ) ) ;
#76728=CARTESIAN_POINT ( 'NONE',  ( -21.87173617678286419, -278.3316267423758177, -197.4934392616594607 ) ) ;
#76729=CARTESIAN_POINT ( 'NONE',  ( -104.7504358689854769, -274.1468479304457446, -241.1944732930645614 ) ) ;
#76730=CARTESIAN_POINT ( 'NONE',  ( -4.066171927379444107, -273.0570839051138137, -201.5619417268292750 ) ) ;
#76731=CARTESIAN_POINT ( 'NONE',  ( -109.8595781668697668, -298.1411517136421594, -257.8498317690542194 ) ) ;
#76733=CARTESIAN_POINT ( 'NONE',  ( -63.14596986960387426, -298.5102405101060299, -201.8477373004160995 ) ) ;
#76735=CARTESIAN_POINT ( 'NONE',  ( 11.33375771337099813, -286.4014152028009335, -327.8859526523521595 ) ) ;
#76736=CARTESIAN_POINT ( 'NONE',  ( -34.47993613328235796, -298.0889596179500245, -197.3611180422582549 ) ) ;
#76737=CARTESIAN_POINT ( 'NONE',  ( 14.60370856817763041, -288.3451503552590225, -327.2723938430602857 ) ) ;
#76738=CARTESIAN_POINT ( 'NONE',  ( -6.932185464183433510, -288.3306037057610638, -341.0931429864613733 ) ) ;
#76739=CARTESIAN_POINT ( 'NONE',  ( -105.0467918063214654, -298.9661115425412277, -237.2789874499145526 ) ) ;
#76740=CARTESIAN_POINT ( 'NONE',  ( 33.26148161316621810, -291.8757249210775626, -295.3197334483541567 ) ) ;
#76741=CARTESIAN_POINT ( 'NONE',  ( 37.98522367718763348, -280.9393962618596561, -285.5273096958051156 ) ) ;
#76743=CARTESIAN_POINT ( 'NONE',  ( -98.79400081414873114, -277.1358528567157578, -227.3435465148481569 ) ) ;
#76745=CARTESIAN_POINT ( 'NONE',  ( -78.40922887016004950, -288.4130594546452926, -331.2547748475975595 ) ) ;
#76748=CARTESIAN_POINT ( 'NONE',  ( -108.8669602638945832, -288.2588691536116698, -293.0971604383435078 ) ) ;
#76749=CARTESIAN_POINT ( 'NONE',  ( -40.57317446955623552, -299.6110061150338879, -196.6192111055412681 ) ) ;
#76750=CARTESIAN_POINT ( 'NONE',  ( 36.02881530851531267, -282.7072136894717005, -248.9747617690478876 ) ) ;
#76751=CARTESIAN_POINT ( 'NONE',  ( -34.80262803020576712, -296.1038995947365606, -195.0067612199095777 ) ) ;
#76752=CARTESIAN_POINT ( 'NONE',  ( -51.01789745730554415, -283.2316833417682460, -342.1201670036364817 ) ) ;
#76753=CARTESIAN_POINT ( 'NONE',  ( 13.89399614490957369, -276.2135002198470488, -217.5380326527090915 ) ) ;
#76754=CARTESIAN_POINT ( 'NONE',  ( 34.53022114635317052, -276.1749785405036732, -256.6852757898665800 ) ) ;
#76755=CARTESIAN_POINT ( 'NONE',  ( 36.41388865671829222, -285.8419503763049079, -286.8343437386976689 ) ) ;
#76756=CARTESIAN_POINT ( 'NONE',  ( -27.60581441161320981, -284.9287777069334311, -344.7784973596588998 ) ) ;
#76757=CARTESIAN_POINT ( 'NONE',  ( -94.00858999500484003, -272.1287512492044698, -223.8324658957658926 ) ) ;
#76759=CARTESIAN_POINT ( 'NONE',  ( 204.9737444410070566, 294.0971962920011720, -54.00000000001803357 ) ) ;
#76760=CARTESIAN_POINT ( 'NONE',  ( 4.225512895823866799, -294.3420781106043478, -335.2403015338224463 ) ) ;
#76761=CARTESIAN_POINT ( 'NONE',  ( -68.25129945820560806, -287.6240421843597801, -202.4167033829201614 ) ) ;
#76763=CARTESIAN_POINT ( 'NONE',  ( 36.57525178469694538, -273.4809262143061233, -305.9938812882205070 ) ) ;
#76764=CARTESIAN_POINT ( 'NONE',  ( -96.93565459347829005, -277.0968812586236822, -318.8865642467521297 ) ) ;
#76765=CARTESIAN_POINT ( 'NONE',  ( -112.5734979646407510, -288.7990036975851922, -282.4696691000957571 ) ) ;
#76766=CARTESIAN_POINT ( 'NONE',  ( -4.500960683627558190, -284.1313966059612994, -336.3322752199168804 ) ) ;
#76767=CARTESIAN_POINT ( 'NONE',  ( -48.74211185284015357, -278.9593193771763708, -343.5432709503215847 ) ) ;
#76768=CARTESIAN_POINT ( 'NONE',  ( -91.99948166029207641, -285.2392658024552929, -323.7571216752605778 ) ) ;
#76769=CARTESIAN_POINT ( 'NONE',  ( -108.8154649949730697, -283.1274117683187797, -287.1083383910242901 ) ) ;
#76770=CARTESIAN_POINT ( 'NONE',  ( -34.25585668506585790, -282.0910847014805540, -195.4117360488422435 ) ) ;
#76771=CARTESIAN_POINT ( 'NONE',  ( -3.828025083772701009, -274.6487784333672835, -201.0224899149199018 ) ) ;
#76772=CARTESIAN_POINT ( 'NONE',  ( -45.65172708368776000, -276.9878992031458438, -346.9644440313794007 ) ) ;
#76773=CARTESIAN_POINT ( 'NONE',  ( -110.5540224271688032, -298.2972234404227265, -283.8952634451722474 ) ) ;
#76777=CARTESIAN_POINT ( 'NONE',  ( -99.01703812007357897, -294.0983534309256129, -314.4547261793791222 ) ) ;
#76778=CARTESIAN_POINT ( 'NONE',  ( 25.33184142990839405, -274.5425675952747611, -232.7129368582133964 ) ) ;
#76779=CARTESIAN_POINT ( 'NONE',  ( -26.27902803094477235, -299.2672730695208543, -193.6682527258752486 ) ) ;
#76780=CARTESIAN_POINT ( 'NONE',  ( -5.381090812785151556, -288.2386053716709284, -203.5901710489817731 ) ) ;
#76781=CARTESIAN_POINT ( 'NONE',  ( -83.74806696574948717, -297.1958651192277330, -331.0012908657889739 ) ) ;
#76782=CARTESIAN_POINT ( 'NONE',  ( 36.71663804834218325, -295.0036142221478599, -289.9409868822082217 ) ) ;
#76784=CARTESIAN_POINT ( 'NONE',  ( -100.3725741073241267, -292.0079916845918433, -310.6989085909413575 ) ) ;
#76785=CARTESIAN_POINT ( 'NONE',  ( -96.21785295733651822, -277.1875605780452361, -224.1493017826633718 ) ) ;
#76786=CARTESIAN_POINT ( 'NONE',  ( -109.8841469871321834, -280.2555290125474698, -287.1180563634273994 ) ) ;
#76787=CARTESIAN_POINT ( 'NONE',  ( -108.9954257056843971, -294.3704572154069865, -290.5367917098691350 ) ) ;
#76788=CARTESIAN_POINT ( 'NONE',  ( -98.77282794680859013, -285.8139437521036825, -314.7942429699178319 ) ) ;
#76789=CARTESIAN_POINT ( 'NONE',  ( -6.875550828619760857, -285.3819894538563631, -203.6687007221675856 ) ) ;
#76790=CARTESIAN_POINT ( 'NONE',  ( 201.4006444668590348, 287.9081297433514806, -97.31964668604067015 ) ) ;
#76792=CARTESIAN_POINT ( 'NONE',  ( -95.78031251298627069, -284.8332872889211558, -226.5773759157260940 ) ) ;
#76794=CARTESIAN_POINT ( 'NONE',  ( 22.62497065170372323, -281.9889408704189009, -222.5334370499905674 ) ) ;
#76795=CARTESIAN_POINT ( 'NONE',  ( -63.31821001435073981, -274.0374721145117292, -202.1031448226012230 ) ) ;
#76796=CARTESIAN_POINT ( 'NONE',  ( -54.85882837433268122, -284.6267097088638707, -195.7879395906978175 ) ) ;
#76797=CARTESIAN_POINT ( 'NONE',  ( 32.95266403754042983, -282.0987973680323080, -239.5143583656991098 ) ) ;
#76799=CARTESIAN_POINT ( 'NONE',  ( -25.52224719976205947, -281.7202806909519950, -194.9753880085647495 ) ) ;
#76800=CARTESIAN_POINT ( 'NONE',  ( 1.315543883392145563, -281.2054010817063840, -203.8254613743454797 ) ) ;
#76801=CARTESIAN_POINT ( 'NONE',  ( 17.40634833298269157, -290.4094976428775112, -226.7417163044926838 ) ) ;
#76802=CARTESIAN_POINT ( 'NONE',  ( -21.25639653131470297, -108.7475251564685976, -362.7871151475208649 ) ) ;
#76804=CARTESIAN_POINT ( 'NONE',  ( -57.37634452483914771, -275.7932986035743284, -198.2054673961312972 ) ) ;
#76805=CARTESIAN_POINT ( 'NONE',  ( -108.2462866289636025, -261.9720010280532279, -317.4642910659676431 ) ) ;
#76806=CARTESIAN_POINT ( 'NONE',  ( 35.54105161292097392, -279.7802643882178586, -286.4841234598790720 ) ) ;
#76807=CARTESIAN_POINT ( 'NONE',  ( 34.48727884711513525, -294.9938061797964224, -245.4114250490830784 ) ) ;
#76809=CARTESIAN_POINT ( 'NONE',  ( -23.50766485369321046, -294.2193438462166455, -342.1937946107894390 ) ) ;
#76810=CARTESIAN_POINT ( 'NONE',  ( -68.29824766140912118, -291.1639872345078288, -199.9108414600736694 ) ) ;
#76812=CARTESIAN_POINT ( 'NONE',  ( -113.7198779826033501, -295.1724553898970385, -266.7449246467346029 ) ) ;
#76813=CARTESIAN_POINT ( 'NONE',  ( 12.68327238162940951, -286.7408048212066660, -324.6886510975755868 ) ) ;
#76814=CARTESIAN_POINT ( 'NONE',  ( 25.88773120472323797, -294.8841451944440450, -231.3675062999054433 ) ) ;
#76815=CARTESIAN_POINT ( 'NONE',  ( -92.02082268316372904, -285.1690072359671717, -319.4864341692789935 ) ) ;
#76817=CARTESIAN_POINT ( 'NONE',  ( -70.80600167280040580, -292.5626899446709785, -201.2745003467363176 ) ) ;
#76818=CARTESIAN_POINT ( 'NONE',  ( 7.836929599663928769, -282.9084735145201535, -327.8441974752027477 ) ) ;
#76819=CARTESIAN_POINT ( 'NONE',  ( -106.8127544581925008, -294.9318585821474130, -302.6377554736166644 ) ) ;
#76820=CARTESIAN_POINT ( 'NONE',  ( -96.26064320211381187, -290.6895856249560097, -319.7041034888595732 ) ) ;
#76821=CARTESIAN_POINT ( 'NONE',  ( -36.38543624903908125, -292.5561848099704321, -193.4155772456277020 ) ) ;
#76822=CARTESIAN_POINT ( 'NONE',  ( 35.45207718627528948, -287.7995411981529514, -276.4792224299424106 ) ) ;
#76825=CARTESIAN_POINT ( 'NONE',  ( -78.78124554001236390, -297.4645748580605300, -333.7887898217801990 ) ) ;
#76826=CARTESIAN_POINT ( 'NONE',  ( -95.18717095392101157, -295.9184518941388546, -220.2101266073456145 ) ) ;
#76827=CARTESIAN_POINT ( 'NONE',  ( -66.15125742854300483, -278.7243331120811831, -203.0167755575455999 ) ) ;
#76829=CARTESIAN_POINT ( 'NONE',  ( 37.22713366733128026, -274.8225227298822801, -251.4134022930541903 ) ) ;
#76830=CARTESIAN_POINT ( 'NONE',  ( -109.7230384929604838, -295.2138079905083146, -256.4502442199338930 ) ) ;
#76831=CARTESIAN_POINT ( 'NONE',  ( -62.18117992897023072, -279.2389104878173498, -340.3719310740302149 ) ) ;
#76832=CARTESIAN_POINT ( 'NONE',  ( 30.21987882562623895, -273.2824364716808532, -239.4747143198748631 ) ) ;
#76833=CARTESIAN_POINT ( 'NONE',  ( -53.22040793449946960, -296.4652670279565996, -342.0722775561085314 ) ) ;
#76834=CARTESIAN_POINT ( 'NONE',  ( -98.71385353567241339, -298.1862380762077009, -230.1732849842972826 ) ) ;
#76836=CARTESIAN_POINT ( 'NONE',  ( -91.08587157039625026, -298.9040373189471325, -216.3425614445917233 ) ) ;
#76837=CARTESIAN_POINT ( 'NONE',  ( -35.50162904485573989, -296.0749791115317748, -195.1950682159290125 ) ) ;
#76838=CARTESIAN_POINT ( 'NONE',  ( 4.555284104978047033, -293.2854069631762286, -210.3946854649783518 ) ) ;
#76839=CARTESIAN_POINT ( 'NONE',  ( -110.3765128903326058, -289.0088883758375573, -279.3772724642715843 ) ) ;
#76841=CARTESIAN_POINT ( 'NONE',  ( 1.159191600861030347, -275.0441616628350516, -203.7334727181245171 ) ) ;
#76842=CARTESIAN_POINT ( 'NONE',  ( -52.64366058546358573, -298.1840897786422033, -198.9093746060461569 ) ) ;
#76843=CARTESIAN_POINT ( 'NONE',  ( -87.84811519967756510, -281.3301567154842928, -214.4369833275779627 ) ) ;
#76844=CARTESIAN_POINT ( 'NONE',  ( -74.05416154775977589, -282.2138878511605640, -337.5432072027315371 ) ) ;
#76845=CARTESIAN_POINT ( 'NONE',  ( -42.80721410208891342, -276.4680116714912970, -347.0647094475549466 ) ) ;
#76846=CARTESIAN_POINT ( 'NONE',  ( -105.7122109433169470, -284.0962294726536470, -244.3212451426253438 ) ) ;
#76847=CARTESIAN_POINT ( 'NONE',  ( 35.75931287015413318, -279.7768593501419900, -287.9165212345840246 ) ) ;
#76848=CARTESIAN_POINT ( 'NONE',  ( -92.44744532713963281, -271.8181609291914924, -221.5888741949748351 ) ) ;
#76849=CARTESIAN_POINT ( 'NONE',  ( -92.96718084120462322, -279.8506860439898674, -320.6871905074064557 ) ) ;
#76853=CARTESIAN_POINT ( 'NONE',  ( -48.79482848485816504, -296.1482044836258751, -195.1895873448658563 ) ) ;
#76854=CARTESIAN_POINT ( 'NONE',  ( 9.406271242195954230, -278.4119172539650435, -329.2889255606859251 ) ) ;
#76855=CARTESIAN_POINT ( 'NONE',  ( -60.05780265172333543, -271.7577189249084881, -198.8296289754283919 ) ) ;
#76857=CARTESIAN_POINT ( 'NONE',  ( -112.1697510040013270, -286.3338913703030926, -281.2215909911712401 ) ) ;
#76861=CARTESIAN_POINT ( 'NONE',  ( 21.09807492070249779, -286.1990395094103974, -317.3896012640129243 ) ) ;
#76863=CARTESIAN_POINT ( 'NONE',  ( -61.15643401280885172, -294.1631289167759178, -339.8411284280082327 ) ) ;
#76864=CARTESIAN_POINT ( 'NONE',  ( 35.78831485485306985, -285.5224157997286056, -257.3087225269305236 ) ) ;
#76865=CARTESIAN_POINT ( 'NONE',  ( 24.80950920047307307, -22.49099280560490399, -345.4124233396505019 ) ) ;
#76866=CARTESIAN_POINT ( 'NONE',  ( -96.86112658669014763, -295.1771302669549186, -224.7064573417206077 ) ) ;
#76867=CARTESIAN_POINT ( 'NONE',  ( -85.06409488138612573, -283.8868155852132418, -210.8188574452699982 ) ) ;
#76868=CARTESIAN_POINT ( 'NONE',  ( 24.81511520159434880, -283.6978039692119182, -310.2416662723389891 ) ) ;
#76869=CARTESIAN_POINT ( 'NONE',  ( 36.69531954020453668, -279.5746205710122467, -253.2014265372545196 ) ) ;
#76870=CARTESIAN_POINT ( 'NONE',  ( -90.59275651568300702, -289.8329213021414716, -320.3681424121349437 ) ) ;
#76871=CARTESIAN_POINT ( 'NONE',  ( -9.037352862421002442, -281.8550182730632514, -202.4329291076968218 ) ) ;
#76872=CARTESIAN_POINT ( 'NONE',  ( 22.23906847704920509, -281.7631645236373288, -227.9025059038118854 ) ) ;
#76873=CARTESIAN_POINT ( 'NONE',  ( 13.51269787187153248, -290.3247237891447412, -326.0397357310200732 ) ) ;
#76875=CARTESIAN_POINT ( 'NONE',  ( -113.5443057820701824, -272.6949299969889466, -258.9447185789064747 ) ) ;
#76876=CARTESIAN_POINT ( 'NONE',  ( -99.46591255800603903, -291.9699541887025589, -311.7658821380492782 ) ) ;
#76878=CARTESIAN_POINT ( 'NONE',  ( -2.602324593224680793, -291.1233781216987495, -342.4248175857292154 ) ) ;
#76880=CARTESIAN_POINT ( 'NONE',  ( -26.07062376046305374, -274.9087881590091911, -344.6779482554795209 ) ) ;
#76882=CARTESIAN_POINT ( 'NONE',  ( -81.42565569830419747, -294.0402114871855588, -332.5789765780154426 ) ) ;
#76883=CARTESIAN_POINT ( 'NONE',  ( -37.14315381731567101, -297.5623635274440630, -197.2967449215204851 ) ) ;
#76884=CARTESIAN_POINT ( 'NONE',  ( -29.07631924951236257, -290.4656279022099170, -343.5894678942593714 ) ) ;
#76885=CARTESIAN_POINT ( 'NONE',  ( 6.206154487261058783, -284.2119424452542944, -330.2072404097167464 ) ) ;
#76886=CARTESIAN_POINT ( 'NONE',  ( -72.92952254726509409, -290.8287756716216563, -338.1017349535645735 ) ) ;
#76887=CARTESIAN_POINT ( 'NONE',  ( -1.245591803044596935, -288.5307547965683170, -204.5603923112500979 ) ) ;
#76888=CARTESIAN_POINT ( 'NONE',  ( -42.43217316056491484, -280.1562955310649272, -193.5295678952614935 ) ) ;
#76889=CARTESIAN_POINT ( 'NONE',  ( -111.4710981498404294, -294.8193518280380658, -255.6609399110392076 ) ) ;
#76890=CARTESIAN_POINT ( 'NONE',  ( -97.17373675951814960, -283.7352074409558895, -318.8496363182581490 ) ) ;
#76891=CARTESIAN_POINT ( 'NONE',  ( 24.81499666903957646, -276.8594682637530582, -229.7728127305347527 ) ) ;
#76893=CARTESIAN_POINT ( 'NONE',  ( 7.450504543161046378, -278.9090924074131408, -326.4764044574609443 ) ) ;
#76894=CARTESIAN_POINT ( 'NONE',  ( 34.77543551412834688, -273.4847523464841288, -246.2557507969009691 ) ) ;
#76896=CARTESIAN_POINT ( 'NONE',  ( -3.114716986823207190, -280.0247965234529488, -205.7984802966873303 ) ) ;
#76897=CARTESIAN_POINT ( 'NONE',  ( -79.99230248998082971, -278.8200339340047549, -334.0562051560213490 ) ) ;
#76898=CARTESIAN_POINT ( 'NONE',  ( -30.89164117063817727, -285.1905093387615011, -193.8546159905229729 ) ) ;
#76899=CARTESIAN_POINT ( 'NONE',  ( 0.4068617851011501196, -294.3226974174677935, -206.6977840534921427 ) ) ;
#76900=CARTESIAN_POINT ( 'NONE',  ( 35.81202702478421429, -276.8798626843932311, -248.8468140989682809 ) ) ;
#76901=CARTESIAN_POINT ( 'NONE',  ( -1.547143709048898197, -275.8317809596364327, -202.7441969895050136 ) ) ;
#76903=CARTESIAN_POINT ( 'NONE',  ( 28.02955897725547274, -275.8273870376234527, -302.9650418396694249 ) ) ;
#76904=CARTESIAN_POINT ( 'NONE',  ( -111.1675064573201439, -298.3948235758292640, -282.5995307722490679 ) ) ;
#76905=CARTESIAN_POINT ( 'NONE',  ( -30.33487976723781543, -284.1406878903274560, -195.8044598530479163 ) ) ;
#76906=CARTESIAN_POINT ( 'NONE',  ( 19.40294650657618192, -292.5110035160992084, -218.3439153488016871 ) ) ;
#76907=CARTESIAN_POINT ( 'NONE',  ( 17.72796013400181181, -274.2794206241090365, -320.7704447901696199 ) ) ;
#76908=CARTESIAN_POINT ( 'NONE',  ( -3.398592021914435435, -290.2117115917122305, -338.5980691811682277 ) ) ;
#76909=CARTESIAN_POINT ( 'NONE',  ( -22.66536255689516466, -291.1647678147143097, -198.5361140622206619 ) ) ;
#76911=CARTESIAN_POINT ( 'NONE',  ( -11.33658538402526084, -290.9590391734051309, -198.4560753402803925 ) ) ;
#76912=CARTESIAN_POINT ( 'NONE',  ( -93.45336087039868289, -290.8818502863744584, -223.6129249373564392 ) ) ;
#76914=CARTESIAN_POINT ( 'NONE',  ( 39.26803746374337578, -288.5748367620718113, -265.8229276596409250 ) ) ;
#76915=CARTESIAN_POINT ( 'NONE',  ( -74.52020881422305365, -279.8764855438762993, -207.4551977821039088 ) ) ;
#76917=CARTESIAN_POINT ( 'NONE',  ( -3.378095802159524652, -293.5346380217991964, -339.1358694524066664 ) ) ;
#76918=CARTESIAN_POINT ( 'NONE',  ( -109.8838510317794004, -285.5258425320400306, -244.8474132593927095 ) ) ;
#76919=CARTESIAN_POINT ( 'NONE',  ( 38.00193571307701745, -287.6871997286742157, -254.5150156346946346 ) ) ;
#76921=CARTESIAN_POINT ( 'NONE',  ( 13.94255196412528619, -282.6418006494040469, -322.4132055708257667 ) ) ;
#76922=CARTESIAN_POINT ( 'NONE',  ( 64.96643722983849045, 47.89135711549346297, -318.9769533625240570 ) ) ;
#76923=CARTESIAN_POINT ( 'NONE',  ( 63.56526613329861419, 48.20594201903070797, -317.9086331218617829 ) ) ;
#76924=CARTESIAN_POINT ( 'NONE',  ( -106.4423271607811898, -259.7000258358197584, -315.5468887844339179 ) ) ;
#76925=CARTESIAN_POINT ( 'NONE',  ( 35.76273596723413561, -274.8015758187369215, -274.3315634204191724 ) ) ;
#76926=CARTESIAN_POINT ( 'NONE',  ( 30.55916282461592459, -274.8427078849937288, -298.1312310828664067 ) ) ;
#76927=CARTESIAN_POINT ( 'NONE',  ( -91.58769398147823892, -296.8118990018231784, -215.8001515871295055 ) ) ;
#76928=CARTESIAN_POINT ( 'NONE',  ( 203.5338562182570001, 292.0436489450776207, -53.99999999998835420 ) ) ;
#76929=CARTESIAN_POINT ( 'NONE',  ( 23.25258900297250975, -273.6094030875871681, -223.6318617462921168 ) ) ;
#76930=CARTESIAN_POINT ( 'NONE',  ( -49.05764131074640488, -275.6611343120919173, -197.2290659742096750 ) ) ;
#76932=CARTESIAN_POINT ( 'NONE',  ( -76.28764799197409729, -274.6243320108757189, -204.2338312892161696 ) ) ;
#76933=CARTESIAN_POINT ( 'NONE',  ( 22.80412073339321211, -288.6219400024127708, -311.8617054626722052 ) ) ;
#76934=CARTESIAN_POINT ( 'NONE',  ( -97.27504928186945676, -296.7091223177130814, -318.4667847877851159 ) ) ;
#76935=CARTESIAN_POINT ( 'NONE',  ( -114.2484962686692285, -297.0897662265755343, -266.7444304478437971 ) ) ;
#76936=CARTESIAN_POINT ( 'NONE',  ( -4.834986371183608966, -292.6592369659877022, -204.9842562496372125 ) ) ;
#76938=CARTESIAN_POINT ( 'NONE',  ( 33.85256884787933984, -277.7996115248241722, -295.8273437185206376 ) ) ;
#76940=CARTESIAN_POINT ( 'NONE',  ( -25.39895610655716851, -279.7081356066872786, -194.3552118414999939 ) ) ;
#76942=CARTESIAN_POINT ( 'NONE',  ( -93.77971946704622042, -278.8336875194699473, -317.0515070767875727 ) ) ;
#76943=CARTESIAN_POINT ( 'NONE',  ( 0.5612836321380542115, -278.3147380947766010, -336.2792770800451194 ) ) ;
#76944=CARTESIAN_POINT ( 'NONE',  ( -112.7317043466922399, -276.5929248515249697, -268.7438369969278256 ) ) ;
#76945=CARTESIAN_POINT ( 'NONE',  ( -35.82122951370943298, -298.7230955458567792, -197.2590104329121345 ) ) ;
#76946=CARTESIAN_POINT ( 'NONE',  ( -45.17132622571710243, -293.7278318508057282, -343.5835260978550423 ) ) ;
#76948=CARTESIAN_POINT ( 'NONE',  ( 21.01532648003455250, -281.3669807022101850, -220.2014386207109169 ) ) ;
#76949=CARTESIAN_POINT ( 'NONE',  ( -109.6221191285575571, -278.8583394546413388, -259.7857695774932836 ) ) ;
#76950=CARTESIAN_POINT ( 'NONE',  ( -62.61664176052439501, -288.0590141791712426, -342.6284718934915077 ) ) ;
#76951=CARTESIAN_POINT ( 'NONE',  ( -105.0489245893652566, -274.9768893035542305, -238.1007335866977996 ) ) ;
#76953=CARTESIAN_POINT ( 'NONE',  ( -34.58213057077002617, -288.2138975673685195, -343.5202244982656907 ) ) ;
#76954=CARTESIAN_POINT ( 'NONE',  ( -39.71153009679694179, -278.2618745588158617, -196.3730369288573456 ) ) ;
#76955=CARTESIAN_POINT ( 'NONE',  ( -66.28486608250479151, -278.2403910190682268, -202.6889043120860094 ) ) ;
#76956=CARTESIAN_POINT ( 'NONE',  ( -26.55786663609574916, -280.9938753476183706, -344.0681837657413666 ) ) ;
#76957=CARTESIAN_POINT ( 'NONE',  ( -90.85243905842411039, -287.2935666412539604, -217.7371416735708181 ) ) ;
#76958=CARTESIAN_POINT ( 'NONE',  ( -87.81475920902107646, -280.5331210238073254, -217.0029608360344753 ) ) ;
#76960=CARTESIAN_POINT ( 'NONE',  ( -87.33576820686256781, -293.3551532516469820, -214.4541076612754296 ) ) ;
#76961=CARTESIAN_POINT ( 'NONE',  ( -53.93212986229021055, -275.5020100719474385, -344.5684756188985602 ) ) ;
#76962=CARTESIAN_POINT ( 'NONE',  ( -53.96906400489967837, -277.9225782758521177, -341.5991676687450536 ) ) ;
#76963=CARTESIAN_POINT ( 'NONE',  ( -55.24034981963281155, -285.2820377730427595, -343.3656847075271799 ) ) ;
#76965=CARTESIAN_POINT ( 'NONE',  ( -105.2091565635610806, -292.0362512703659945, -303.6962708431841520 ) ) ;
#76966=CARTESIAN_POINT ( 'NONE',  ( -80.93773930535884631, -293.6434239255821126, -331.4519757971451099 ) ) ;
#76967=CARTESIAN_POINT ( 'NONE',  ( 27.00812565924913500, -286.1965218845581376, -228.3699434157463486 ) ) ;
#76969=CARTESIAN_POINT ( 'NONE',  ( 21.88849600603380452, -273.6314953436670976, -226.8521839007555343 ) ) ;
#76970=CARTESIAN_POINT ( 'NONE',  ( 33.92952733776302665, -291.9624114762742693, -291.1739805902424223 ) ) ;
#76972=CARTESIAN_POINT ( 'NONE',  ( -111.9578785049571223, -289.2343554908222814, -254.3266412939698000 ) ) ;
#76973=CARTESIAN_POINT ( 'NONE',  ( -30.47694198535674559, -287.7403961922369717, -196.8297286551571972 ) ) ;
#76974=CARTESIAN_POINT ( 'NONE',  ( 25.53167739099729516, -285.2216615680111431, -227.6657143534044110 ) ) ;
#76976=CARTESIAN_POINT ( 'NONE',  ( -109.2923710593129840, -285.7745612175551173, -285.8635637361780937 ) ) ;
#76978=CARTESIAN_POINT ( 'NONE',  ( -89.78572593098405719, -286.0916735583547847, -219.2763901724217135 ) ) ;
#76979=CARTESIAN_POINT ( 'NONE',  ( 34.80249007755185886, -295.8132040623688113, -292.3009547389195291 ) ) ;
#76981=CARTESIAN_POINT ( 'NONE',  ( 9.611743351465115381, -274.4922335098502231, -329.6283208015555033 ) ) ;
#76982=CARTESIAN_POINT ( 'NONE',  ( 38.71553715295499387, -276.0381860407999852, -282.5718503297363213 ) ) ;
#76983=CARTESIAN_POINT ( 'NONE',  ( -30.79715606001322215, -290.2139746343372622, -195.0333000752978592 ) ) ;
#76984=CARTESIAN_POINT ( 'NONE',  ( -110.5496847997783476, -278.8543007676240109, -246.3257844339869962 ) ) ;
#76985=CARTESIAN_POINT ( 'NONE',  ( -96.90184065772848498, -297.9136378316295009, -315.3759034152589606 ) ) ;
#76988=CARTESIAN_POINT ( 'NONE',  ( -19.68124197500630501, -284.9688554521978290, -199.0214257039185100 ) ) ;
#76989=CARTESIAN_POINT ( 'NONE',  ( 22.17613448769722240, -278.9268243360425004, -224.7043097940381529 ) ) ;
#76991=CARTESIAN_POINT ( 'NONE',  ( 38.44658308318671658, -274.1496698841874036, -279.6825883453341817 ) ) ;
#76992=CARTESIAN_POINT ( 'NONE',  ( -36.47327549706410110, -276.3896055142875525, -343.4703777290328048 ) ) ;
#76993=CARTESIAN_POINT ( 'NONE',  ( 19.37902799195334680, -295.7332439217461797, -317.4086126645106560 ) ) ;
#76994=CARTESIAN_POINT ( 'NONE',  ( 39.10468502056978934, -280.3956473024632601, -264.2420733834683801 ) ) ;
#76995=CARTESIAN_POINT ( 'NONE',  ( -38.33349419775058209, -296.0061404914874856, -343.5896970578966716 ) ) ;
#76996=CARTESIAN_POINT ( 'NONE',  ( -32.02992129025761869, -296.3016590936503576, -346.6965208343950735 ) ) ;
#76997=CARTESIAN_POINT ( 'NONE',  ( -75.20882932078620797, -297.3658662381225781, -207.8919318826508800 ) ) ;
#76998=CARTESIAN_POINT ( 'NONE',  ( -60.91100295596007186, -293.7465757119263117, -199.1062761145201989 ) ) ;
#76999=CARTESIAN_POINT ( 'NONE',  ( -63.20343213100047564, -285.8910563097514341, -197.8340828693793583 ) ) ;
#77000=CARTESIAN_POINT ( 'NONE',  ( 9.739654017775013273, -274.5519620265484377, -329.7884476712060291 ) ) ;
#77001=CARTESIAN_POINT ( 'NONE',  ( 35.07174509385883709, -287.7178248370943834, -296.6943353081996975 ) ) ;
#77002=CARTESIAN_POINT ( 'NONE',  ( -96.10090313381023464, -281.1669683924969263, -224.3057348175780419 ) ) ;
#77004=CARTESIAN_POINT ( 'NONE',  ( 33.61952280722571373, -286.3720464971211754, -252.2020916793732965 ) ) ;
#77005=CARTESIAN_POINT ( 'NONE',  ( -41.90611935587904924, -289.9944572538296939, -195.5001353075423083 ) ) ;
#77007=CARTESIAN_POINT ( 'NONE',  ( 81.08292338999881110, 82.25620239566015357, -296.3357184930298445 ) ) ;
#77008=CARTESIAN_POINT ( 'NONE',  ( 35.71665683933490243, -287.0687889237887020, -271.0429674359417049 ) ) ;
#77010=CARTESIAN_POINT ( 'NONE',  ( 15.59995472104877301, -283.2660809251399883, -325.9488989629570028 ) ) ;
#77011=CARTESIAN_POINT ( 'NONE',  ( -105.7888645952828597, -290.0610408584786910, -235.4904470152518456 ) ) ;
#77012=CARTESIAN_POINT ( 'NONE',  ( 23.93614727145840959, -282.5439933668443473, -225.0680077438634612 ) ) ;
#77013=CARTESIAN_POINT ( 'NONE',  ( -9.059085678266479036, -281.7295696065875177, -199.2739039927778322 ) ) ;
#77014=CARTESIAN_POINT ( 'NONE',  ( 17.06422943565276285, -280.6891292655526513, -221.6887969692598688 ) ) ;
#77015=CARTESIAN_POINT ( 'NONE',  ( 34.82919090812784901, -277.8154144086593647, -290.8131523905287281 ) ) ;
#77016=CARTESIAN_POINT ( 'NONE',  ( -39.10783922643397403, -295.0737427575077731, -347.3408604651460792 ) ) ;
#77017=CARTESIAN_POINT ( 'NONE',  ( -112.0125344030138450, -288.5976342690941010, -268.3938059634269280 ) ) ;
#77018=CARTESIAN_POINT ( 'NONE',  ( -110.7382015680781535, -271.3832025871527094, -267.6071348884254917 ) ) ;
#77020=CARTESIAN_POINT ( 'NONE',  ( -87.88906082301696188, -285.6850755159490518, -325.0784697405596830 ) ) ;
#77021=CARTESIAN_POINT ( 'NONE',  ( -64.14522180977439803, -296.4734619401404530, -342.2155801616106032 ) ) ;
#77022=CARTESIAN_POINT ( 'NONE',  ( -73.84050084666280611, -284.2016409813550695, -333.7570198402976303 ) ) ;
#77024=CARTESIAN_POINT ( 'NONE',  ( 28.30756358580422472, -274.0888206018845494, -230.4726114452056720 ) ) ;
#77025=CARTESIAN_POINT ( 'NONE',  ( -114.0101373136554770, -291.1210124710574405, -276.9531225384577056 ) ) ;
#77026=CARTESIAN_POINT ( 'NONE',  ( -84.72173070950167073, -283.5465763757330251, -211.2388871393937961 ) ) ;
#77027=CARTESIAN_POINT ( 'NONE',  ( 29.45518768648751973, -293.3881812978008838, -232.0999095627983877 ) ) ;
#77028=CARTESIAN_POINT ( 'NONE',  ( 20.37678908275908896, -288.5154087295122167, -315.1101416684124956 ) ) ;
#77030=CARTESIAN_POINT ( 'NONE',  ( -69.88240323175847379, -196.0786339892123635, -356.6774816750892114 ) ) ;
#77031=CARTESIAN_POINT ( 'NONE',  ( 0.5411208059672262261, -284.0769505835842210, -336.6151734898739392 ) ) ;
#77032=CARTESIAN_POINT ( 'NONE',  ( -69.85430415644619018, -289.1237833571632905, -202.7746430608542312 ) ) ;
#77034=CARTESIAN_POINT ( 'NONE',  ( 20.41605115271496018, -281.1061830307352807, -315.5083021875493046 ) ) ;
#77035=CARTESIAN_POINT ( 'NONE',  ( -56.92274980391026418, -276.9645806723872852, -344.8629614518559947 ) ) ;
#77036=CARTESIAN_POINT ( 'NONE',  ( -82.41185862518261729, -281.4358380463647222, -210.5573600565763570 ) ) ;
#77037=CARTESIAN_POINT ( 'NONE',  ( -37.46162067202239854, -140.9052193018087848, -362.9178459242288568 ) ) ;
#77038=CARTESIAN_POINT ( 'NONE',  ( 37.10754630562437484, -279.9094352774340564, -253.1013608149115157 ) ) ;
#77039=CARTESIAN_POINT ( 'NONE',  ( -99.46222977079803229, -283.1341647278430855, -228.9740837855790687 ) ) ;
#77040=CARTESIAN_POINT ( 'NONE',  ( -112.9501668877829417, -274.4839910648973387, -264.7418366708396888 ) ) ;
#77041=CARTESIAN_POINT ( 'NONE',  ( 33.36617924567667615, -293.8018475188829939, -251.9658947903538149 ) ) ;
#77043=CARTESIAN_POINT ( 'NONE',  ( -77.51078714589368701, -290.1854006632938194, -208.8169230859111281 ) ) ;
#77044=CARTESIAN_POINT ( 'NONE',  ( -37.11892092752835737, -277.7008061531869885, -347.2719043138369557 ) ) ;
#77045=CARTESIAN_POINT ( 'NONE',  ( 2.929940339339094812, -274.6090749914681055, -209.4139665111396198 ) ) ;
#77046=CARTESIAN_POINT ( 'NONE',  ( -87.82252213641214666, -272.2865916653408931, -212.5568331142568468 ) ) ;
#77048=CARTESIAN_POINT ( 'NONE',  ( -102.5945760320706910, -271.0459574960322016, -233.2837800218109976 ) ) ;
#77052=CARTESIAN_POINT ( 'NONE',  ( 34.63512194200365002, -282.4482011167932001, -256.3823509844918931 ) ) ;
#77053=CARTESIAN_POINT ( 'NONE',  ( 33.64889274247908446, -283.6599195083750828, -297.4592680287849475 ) ) ;
#77054=CARTESIAN_POINT ( 'NONE',  ( -108.5264572406010615, -283.6809846479206385, -287.0478253691944133 ) ) ;
#77055=CARTESIAN_POINT ( 'NONE',  ( -21.74530855578876398, -272.6552654742687309, -198.2279565175680602 ) ) ;
#77056=CARTESIAN_POINT ( 'NONE',  ( 35.26847523724462974, -283.2114244290195870, -254.8530575296113625 ) ) ;
#77057=CARTESIAN_POINT ( 'NONE',  ( 31.77524096876192061, -273.6943458334019965, -244.7963726310247239 ) ) ;
#77059=CARTESIAN_POINT ( 'NONE',  ( -2.780021451133341870, -275.6001369539969232, -205.7103914492528816 ) ) ;
#77061=CARTESIAN_POINT ( 'NONE',  ( -38.17842532867272354, -280.8447442492000619, -193.5271495036795670 ) ) ;
#77064=CARTESIAN_POINT ( 'NONE',  ( -106.8033311858618362, -286.8060493221394154, -239.9744768840502331 ) ) ;
#77065=CARTESIAN_POINT ( 'NONE',  ( 8.320992971831785212, -293.6061957033166436, -327.5884466100519035 ) ) ;
#77066=CARTESIAN_POINT ( 'NONE',  ( -111.4459647421723503, -289.6430735994253496, -290.9006104981398835 ) ) ;
#77067=CARTESIAN_POINT ( 'NONE',  ( 30.90472853489130145, -285.4113809929067997, -241.5856899920826493 ) ) ;
#77068=CARTESIAN_POINT ( 'NONE',  ( -37.26215787424501258, -284.6278565616020160, -196.7593913820396097 ) ) ;
#77069=CARTESIAN_POINT ( 'NONE',  ( -103.3026222840980495, -289.2430941396015101, -236.6749666403671597 ) ) ;
#77070=CARTESIAN_POINT ( 'NONE',  ( -104.4703060873563345, -285.3599628368435788, -300.0407535202740519 ) ) ;
#77071=CARTESIAN_POINT ( 'NONE',  ( -12.55191763875878586, -274.7297834185234819, -341.2002388274104874 ) ) ;
#77072=CARTESIAN_POINT ( 'NONE',  ( 35.92770749046399459, -285.6847741258068254, -249.2443098591791397 ) ) ;
#77073=CARTESIAN_POINT ( 'NONE',  ( -107.9760697139818859, -298.8790747096514906, -245.1463112088183891 ) ) ;
#77074=CARTESIAN_POINT ( 'NONE',  ( 24.06252069718013331, -284.9640712522170247, -226.9851382692413608 ) ) ;
#77075=CARTESIAN_POINT ( 'NONE',  ( 22.29816566643246034, -281.9015615755041608, -227.8582374154853198 ) ) ;
#77076=CARTESIAN_POINT ( 'NONE',  ( 11.25051781303261045, -290.3808272807742696, -327.7093941479237174 ) ) ;
#77079=CARTESIAN_POINT ( 'NONE',  ( -25.11624519921462451, -296.8177311834359102, -344.9785932560251354 ) ) ;
#77080=CARTESIAN_POINT ( 'NONE',  ( -97.19280280957008245, -277.1702440446872515, -225.1419538124783628 ) ) ;
#77081=CARTESIAN_POINT ( 'NONE',  ( 4.063150868354068024, -291.7915996332590112, -205.5694027574573113 ) ) ;
#77082=CARTESIAN_POINT ( 'NONE',  ( -93.33825809041043442, -295.6291448942171201, -222.2706361474565995 ) ) ;
#77083=CARTESIAN_POINT ( 'NONE',  ( 18.34910599065556980, -279.5584106096611663, -222.3857979285616580 ) ) ;
#77084=CARTESIAN_POINT ( 'NONE',  ( 1.382029900557905089, -272.6537274690363688, -206.7860683948709379 ) ) ;
#77085=CARTESIAN_POINT ( 'NONE',  ( 27.91680234231528601, -294.4107225774616836, -236.5591752580010620 ) ) ;
#77086=CARTESIAN_POINT ( 'NONE',  ( -20.25526795762937127, -288.7662352645559736, -195.3538533559490702 ) ) ;
#77087=CARTESIAN_POINT ( 'NONE',  ( -72.93978587911213651, -296.0694712879067652, -202.8084855493224836 ) ) ;
#77088=CARTESIAN_POINT ( 'NONE',  ( 33.49859180651249346, -292.1449242058744176, -297.8497892959048841 ) ) ;
#77090=CARTESIAN_POINT ( 'NONE',  ( -87.11466264322206143, -291.1867083139763963, -324.6338007384335924 ) ) ;
#77092=CARTESIAN_POINT ( 'NONE',  ( -106.7276692892395573, -291.6624126686373302, -247.1622169206927140 ) ) ;
#77094=CARTESIAN_POINT ( 'NONE',  ( -96.07667315357234372, -291.0917637214879505, -319.5567740437876978 ) ) ;
#77095=CARTESIAN_POINT ( 'NONE',  ( -98.46934676353225768, -281.9742560001290599, -314.5144165387331441 ) ) ;
#77096=CARTESIAN_POINT ( 'NONE',  ( 30.82839066351708013, -293.2034134699283641, -244.2490762878700536 ) ) ;
#77097=CARTESIAN_POINT ( 'NONE',  ( -11.50935519425200226, -280.3793842889527923, -197.7676286605547773 ) ) ;
#77098=CARTESIAN_POINT ( 'NONE',  ( -112.1995860153573972, -283.9936799669806078, -288.3624367532527799 ) ) ;
#77099=CARTESIAN_POINT ( 'NONE',  ( -18.02420892919868223, -286.8025241078127010, -342.7120662234895576 ) ) ;
#77100=CARTESIAN_POINT ( 'NONE',  ( -40.30702125146652293, -281.2294074770276211, -344.5370733382084154 ) ) ;
#77101=CARTESIAN_POINT ( 'NONE',  ( -73.42058401816386493, -278.0623772438861465, -203.1077589245088006 ) ) ;
#77102=CARTESIAN_POINT ( 'NONE',  ( -43.62716680474309783, -284.8949647816355082, -193.8751910643043743 ) ) ;
#77104=CARTESIAN_POINT ( 'NONE',  ( 35.63212331641676656, -295.3003208156014239, -281.7059976894473721 ) ) ;
#77105=CARTESIAN_POINT ( 'NONE',  ( 28.59670578578791122, -277.4838392500580539, -308.9711285660002318 ) ) ;
#77106=CARTESIAN_POINT ( 'NONE',  ( -51.28907848291654403, -276.9021381626692460, -342.0378793750112436 ) ) ;
#77107=CARTESIAN_POINT ( 'NONE',  ( -53.39139012624264780, -292.0185859414371521, -194.9978724050712913 ) ) ;
#77108=CARTESIAN_POINT ( 'NONE',  ( -73.60676394207003170, -281.6090055231380234, -336.7079612746338739 ) ) ;
#77110=CARTESIAN_POINT ( 'NONE',  ( 22.00238956904736654, -292.0122295526111884, -227.4249021459777680 ) ) ;
#77111=CARTESIAN_POINT ( 'NONE',  ( -101.4204003466219461, -294.0295443658419572, -309.3344527832240374 ) ) ;
#77114=CARTESIAN_POINT ( 'NONE',  ( 17.12226068605793827, -293.7560628651285697, -319.0797258749728940 ) ) ;
#77115=DIRECTION ( 'NONE',  ( 0.000000000000000000, 0.000000000000000000, -1.000000000000000000 ) ) ;
#77117=CARTESIAN_POINT ( 'NONE',  ( -53.28691492658257545, -283.3380690714490697, -200.3538533559491555 ) ) ;
#77118=CARTESIAN_POINT ( 'NONE',  ( -107.5529561909772696, -296.0095768446936404, -239.1942802845665028 ) ) ;
#77119=CARTESIAN_POINT ( 'NONE',  ( 36.47945019456036420, -279.4743620972552662, -253.2528424591031353 ) ) ;
#77120=CARTESIAN_POINT ( 'NONE',  ( 22.59502564391964796, -288.2266882164058757, -222.7914558966029972 ) ) ;
#77121=CARTESIAN_POINT ( 'NONE',  ( 15.97591771424503371, -286.6679669768500389, -220.4805445411825815 ) ) ;
#77122=CARTESIAN_POINT ( 'NONE',  ( -40.51644187217473103, -278.6128860674530188, -343.9986203765841992 ) ) ;
#77123=CARTESIAN_POINT ( 'NONE',  ( -103.9898223251929892, -295.0198014417298396, -236.6324984908770830 ) ) ;
#77124=CARTESIAN_POINT ( 'NONE',  ( -67.69050609239340588, -297.2160679832949199, -337.8800044027375407 ) ) ;
#77125=CARTESIAN_POINT ( 'NONE',  ( -109.4361949955159616, -277.1655813682788789, -284.1940162291792831 ) ) ;
#77128=CARTESIAN_POINT ( 'NONE',  ( -99.07294091365119471, -296.8309679794263047, -224.3500100255391771 ) ) ;
#77129=CARTESIAN_POINT ( 'NONE',  ( -109.1076462815651951, -292.2138832813661793, -290.3236280021598645 ) ) ;
#77130=CARTESIAN_POINT ( 'NONE',  ( 38.70526900344345478, -295.2230344794398320, -275.9598567637233373 ) ) ;
#77132=CARTESIAN_POINT ( 'NONE',  ( 23.59905060707956181, -288.7632899182822257, -310.7587002622397563 ) ) ;
#77135=CARTESIAN_POINT ( 'NONE',  ( 36.37712711407280608, -280.3410715437157705, -248.9047471710078128 ) ) ;
#77136=CARTESIAN_POINT ( 'NONE',  ( -108.7969599933700664, -297.5661075139699960, -241.8021672348784818 ) ) ;
#77137=CARTESIAN_POINT ( 'NONE',  ( -95.61342889771168529, -289.3537127779962361, -221.9188601416647941 ) ) ;
#77138=CARTESIAN_POINT ( 'NONE',  ( 19.36510139688301990, -299.0772331312804795, -193.3791356014287715 ) ) ;
#77142=CARTESIAN_POINT ( 'NONE',  ( 7.542467614791021013, -289.9726308056318089, -332.1362490203076732 ) ) ;
#77143=CARTESIAN_POINT ( 'NONE',  ( -72.02372285203398405, -295.1237833571632336, -198.2697987213421698 ) ) ;
#77145=CARTESIAN_POINT ( 'NONE',  ( -7.568785372384704502, -279.7809116860776157, -199.4462947077354897 ) ) ;
#77146=CARTESIAN_POINT ( 'NONE',  ( -44.21756429591481208, -287.9651449195740724, -195.8443351868794764 ) ) ;
#77147=CARTESIAN_POINT ( 'NONE',  ( -36.55314179334069280, -284.6366010916459572, -193.9414740894099225 ) ) ;
#77148=CARTESIAN_POINT ( 'NONE',  ( 30.76490094069783154, -273.1427144188515399, -239.2272965527591566 ) ) ;
#77149=CARTESIAN_POINT ( 'NONE',  ( -90.28314482040298117, -275.2160841483324134, -218.0302701873049500 ) ) ;
#77150=CARTESIAN_POINT ( 'NONE',  ( -95.23941597198201237, -287.9830567207312697, -317.1496710895513615 ) ) ;
#77151=CARTESIAN_POINT ( 'NONE',  ( -106.4397080345745792, -280.0077188122627945, -301.5655412829672173 ) ) ;
#77152=CARTESIAN_POINT ( 'NONE',  ( -51.82736042554250844, -279.8617439022426083, -198.7610426472906227 ) ) ;
#77153=CARTESIAN_POINT ( 'NONE',  ( -24.85082918697033705, -279.5643063469011054, -198.3342423664415435 ) ) ;
#77154=CARTESIAN_POINT ( 'NONE',  ( 39.39822674470777741, -276.6417865678998282, -271.1546663137556266 ) ) ;
#77155=CARTESIAN_POINT ( 'NONE',  ( 38.47606365382345217, -280.4846042018306775, -281.3007438277670076 ) ) ;
#77156=CARTESIAN_POINT ( 'NONE',  ( 101.4667014786534196, 115.9046547678812402, -280.3899664935571536 ) ) ;
#77157=CARTESIAN_POINT ( 'NONE',  ( 37.98554189617519228, -276.3079132803979974, -255.5750832655114380 ) ) ;
#77159=CARTESIAN_POINT ( 'NONE',  ( -111.1526627510328495, -274.3190909615437363, -250.8028351022462630 ) ) ;
#77160=CARTESIAN_POINT ( 'NONE',  ( -20.19161114001083490, -285.3376638359844719, -345.3538533559490702 ) ) ;
#77163=CARTESIAN_POINT ( 'NONE',  ( 23.01216766782999201, -289.2091694022353181, -311.9961898519719625 ) ) ;
#77164=CARTESIAN_POINT ( 'NONE',  ( 38.62647161556693476, -289.2910459671626882, -268.6845461064718279 ) ) ;
#77165=CARTESIAN_POINT ( 'NONE',  ( -66.37713829960758005, -288.7911076824233305, -337.5034831519449199 ) ) ;
#77166=CARTESIAN_POINT ( 'NONE',  ( -3.510755920250064666, -285.9944197183993992, -201.2452687273539027 ) ) ;
#77167=CARTESIAN_POINT ( 'NONE',  ( -69.93022918456772175, -196.8786560775615158, -360.4189127159840496 ) ) ;
#77168=CARTESIAN_POINT ( 'NONE',  ( -49.25115757787841630, -278.2977017474166246, -197.5283970617807370 ) ) ;
#77169=CARTESIAN_POINT ( 'NONE',  ( -7.784554799578522477, -288.3040946151819526, -202.2638299135906550 ) ) ;
#77170=CARTESIAN_POINT ( 'NONE',  ( 14.39781181031079704, -280.7886961341544065, -322.9089477586801991 ) ) ;
#77171=CARTESIAN_POINT ( 'NONE',  ( -79.35037821838379557, -280.7867802708560703, -210.0575986654147869 ) ) ;
#77172=CARTESIAN_POINT ( 'NONE',  ( -69.27265456268649757, -277.9762532532120076, -336.0895201065175684 ) ) ;
#77173=CARTESIAN_POINT ( 'NONE',  ( -105.6430817444238386, -289.7972595703521961, -235.5609246756592938 ) ) ;
#77174=CARTESIAN_POINT ( 'NONE',  ( -113.7422162882503187, -285.2523065848033639, -278.5537946324250242 ) ) ;
#77175=CARTESIAN_POINT ( 'NONE',  ( -65.22403631520238321, -283.8992606451167262, -342.0837629013142305 ) ) ;
#77176=CARTESIAN_POINT ( 'NONE',  ( 34.33383619676914833, -281.5353573717350741, -256.4526769708820666 ) ) ;
#77179=CARTESIAN_POINT ( 'NONE',  ( -101.2464683506749026, -291.8692335019797497, -311.1575699743892756 ) ) ;
#77180=CARTESIAN_POINT ( 'NONE',  ( -96.18874809594754538, -289.8988664898998309, -221.4499465881910396 ) ) ;
#77181=CARTESIAN_POINT ( 'NONE',  ( 33.08961400738228065, -274.3442248985718379, -250.1089695721849750 ) ) ;
#77182=CARTESIAN_POINT ( 'NONE',  ( -104.5179047653451363, -295.4136782726236561, -307.8955234835698320 ) ) ;
#77184=CARTESIAN_POINT ( 'NONE',  ( -97.31443254186125102, -289.6257781146932757, -227.4498505701685360 ) ) ;
#77185=CARTESIAN_POINT ( 'NONE',  ( -78.53204535554695553, -293.8545225344570326, -331.9155491757897494 ) ) ;
#77186=CARTESIAN_POINT ( 'NONE',  ( -110.0958104779046209, -291.8893723169344412, -260.2897552016919462 ) ) ;
#77188=CARTESIAN_POINT ( 'NONE',  ( -83.90258770686145340, -291.6913500186184365, -329.2243383782388264 ) ) ;
#77189=CARTESIAN_POINT ( 'NONE',  ( -37.75867566610864401, -290.0467844235909070, -195.1956035315612326 ) ) ;
#77190=CARTESIAN_POINT ( 'NONE',  ( 37.58004250640482269, -295.4957536657421429, -265.9558591376419372 ) ) ;
#77191=CARTESIAN_POINT ( 'NONE',  ( 22.17581839113421083, -287.8978231578880127, -227.6016006015461244 ) ) ;
#77192=CARTESIAN_POINT ( 'NONE',  ( 30.58447879850155360, -295.9762457331753467, -302.6704645818480230 ) ) ;
#77193=CARTESIAN_POINT ( 'NONE',  ( 21.45872483227258698, -276.8867311109390243, -223.2140608393319496 ) ) ;
#77194=CARTESIAN_POINT ( 'NONE',  ( -20.54349816217299818, -297.4546192300558687, -193.5248136303333695 ) ) ;
#77195=CARTESIAN_POINT ( 'NONE',  ( -4.638235026735377353, -274.8552159000870461, -336.7714146947103586 ) ) ;
#77196=CARTESIAN_POINT ( 'NONE',  ( -35.60516676954190274, -278.1539211770402176, -195.9287245098378207 ) ) ;
#77197=CARTESIAN_POINT ( 'NONE',  ( -109.5230369993198991, -273.9353492515585913, -256.7853752516125496 ) ) ;
#77198=CARTESIAN_POINT ( 'NONE',  ( -108.7510992504447245, -298.2107675610492947, -252.5310447746156228 ) ) ;
#77200=CARTESIAN_POINT ( 'NONE',  ( -93.74459404252580441, -298.0142710445006173, -223.7442516318711796 ) ) ;
#77202=CARTESIAN_POINT ( 'NONE',  ( 19.31913756162407125, -286.2592727476167056, -320.0590784737461263 ) ) ;
#77203=CARTESIAN_POINT ( 'NONE',  ( -87.33175687242416529, -273.1651468073987985, -217.0942201121042103 ) ) ;
#77204=CARTESIAN_POINT ( 'NONE',  ( -35.14823699187664374, -286.0789470517875088, -193.3792229723000560 ) ) ;
#77205=CARTESIAN_POINT ( 'NONE',  ( -48.87002248114648495, -288.8617396216693010, -346.5257704025116254 ) ) ;
#77206=CARTESIAN_POINT ( 'NONE',  ( -103.1538531219983668, -298.0445600774226591, -307.1715045660848205 ) ) ;
#77207=CARTESIAN_POINT ( 'NONE',  ( -23.19665252841348391, -292.8708136314868398, -343.8983406446320714 ) ) ;
#77209=CARTESIAN_POINT ( 'NONE',  ( 32.24180987646308694, -281.1689552750741541, -303.0792889612517342 ) ) ;
#77211=CARTESIAN_POINT ( 'NONE',  ( 31.98288692825982693, -290.6237833571633473, -237.0123917617630980 ) ) ;
#77212=CARTESIAN_POINT ( 'NONE',  ( -0.4778554359995536571, -278.5419125565632612, -205.0315369040635574 ) ) ;
#77214=CARTESIAN_POINT ( 'NONE',  ( -63.97923812062445137, -288.2022525483117761, -338.8083807621004553 ) ) ;
#77216=CARTESIAN_POINT ( 'NONE',  ( -106.9792876876985162, -288.1875797798215899, -298.3503455605481349 ) ) ;
#77217=CARTESIAN_POINT ( 'NONE',  ( -86.64976378570321458, -298.9531321934215384, -215.4506884472496040 ) ) ;
#77218=CARTESIAN_POINT ( 'NONE',  ( -10.88885579115580171, -284.1393066052172571, -342.1031320851379292 ) ) ;
#77219=CARTESIAN_POINT ( 'NONE',  ( -74.93695352436466806, -295.5746080074775364, -204.9942468947497218 ) ) ;
#77220=CARTESIAN_POINT ( 'NONE',  ( 30.02149271457893320, -281.1748314979352017, -242.2328359510785845 ) ) ;
#77221=CARTESIAN_POINT ( 'NONE',  ( -102.3175327946302957, -297.2603842766558273, -229.0435530278357419 ) ) ;
#77222=CARTESIAN_POINT ( 'NONE',  ( -48.98642912152735107, -275.3263192974031881, -197.6474684415731247 ) ) ;
#77223=CARTESIAN_POINT ( 'NONE',  ( 32.45361939265070816, -283.1933631698066165, -242.7674620859592665 ) ) ;
#77225=CARTESIAN_POINT ( 'NONE',  ( -108.8333058931776947, -271.6855809578856338, -254.1384061293102548 ) ) ;
#77228=CARTESIAN_POINT ( 'NONE',  ( -95.41729670089114279, -287.1807752485198648, -223.4465878802722330 ) ) ;
#77230=CARTESIAN_POINT ( 'NONE',  ( -99.90806341382575795, -275.4094976428775681, -320.2154176792147382 ) ) ;
#77231=CARTESIAN_POINT ( 'NONE',  ( -97.80818132016572974, -277.1141899951845744, -317.7738111518575579 ) ) ;
#77232=CARTESIAN_POINT ( 'NONE',  ( -105.8038040998388993, -288.5165352701823167, -303.9382687494446031 ) ) ;
#77233=CARTESIAN_POINT ( 'NONE',  ( -69.29241909287274837, -285.0004725045340592, -336.7818214500148883 ) ) ;
#77234=CARTESIAN_POINT ( 'NONE',  ( 31.86149825917260969, -276.8140934790913548, -244.7221291755344055 ) ) ;
#77235=CARTESIAN_POINT ( 'NONE',  ( -113.5655135601975019, -286.0536449265675287, -264.3130900155326231 ) ) ;
#77236=CARTESIAN_POINT ( 'NONE',  ( -33.49065488986707351, -281.7975541347797730, -343.6697340270898735 ) ) ;
#77237=CARTESIAN_POINT ( 'NONE',  ( 10.53417674869039544, -282.7130705968492066, -212.5621547007312699 ) ) ;
#77238=CARTESIAN_POINT ( 'NONE',  ( -13.06449860147223774, -274.5257687079455877, -197.2884316317034745 ) ) ;
#77239=CARTESIAN_POINT ( 'NONE',  ( -9.213795940154822617, -276.5277052220291694, -342.0397131871494594 ) ) ;
#77240=CARTESIAN_POINT ( 'NONE',  ( -53.43737329538826941, -297.1802302930198039, -343.0931690192838914 ) ) ;
#77243=CARTESIAN_POINT ( 'NONE',  ( -81.17667521555783594, -293.7799658324468624, -332.2216527674179360 ) ) ;
#77244=EDGE_CURVE ( 'NONE', #64642, #55253, #72684, .T. ) ;
#77245=CARTESIAN_POINT ( 'NONE',  ( 32.15478393937396362, -275.3586503405441022, -292.9050116996871225 ) ) ;
#77246=CARTESIAN_POINT ( 'NONE',  ( -36.20395713954953010, -299.1457486080698231, -193.6700243703820945 ) ) ;
#77248=CARTESIAN_POINT ( 'NONE',  ( -41.40060480639604634, -287.7605246099691385, -196.4464889012422475 ) ) ;
#77249=CARTESIAN_POINT ( 'NONE',  ( 36.40745503038448305, -294.8242035897088726, -250.7207104913053968 ) ) ;
#77250=CARTESIAN_POINT ( 'NONE',  ( 35.90279891270316170, -294.4740753464654972, -247.9278373721565458 ) ) ;
#77251=CARTESIAN_POINT ( 'NONE',  ( -111.6058545418704142, -292.4337688319313315, -279.5732727291029960 ) ) ;
#77252=CARTESIAN_POINT ( 'NONE',  ( -5.978376501635822571, -278.4651481980118888, -202.4032514162272491 ) ) ;
#77253=CARTESIAN_POINT ( 'NONE',  ( -110.1685977613244916, -280.2729174686764964, -285.7740081200694249 ) ) ;
#77254=CARTESIAN_POINT ( 'NONE',  ( -56.19109979435656044, -293.3765524300336551, -342.4285268525277388 ) ) ;
#77255=CARTESIAN_POINT ( 'NONE',  ( -91.53343208344301729, -285.6743392763380598, -323.3097881022966362 ) ) ;
#77256=CARTESIAN_POINT ( 'NONE',  ( -110.5359407540881591, -283.5372398152482560, -265.4307739675700759 ) ) ;
#77257=CARTESIAN_POINT ( 'NONE',  ( -97.57403984170483113, -248.8065872697612235, -333.5881438307000053 ) ) ;
#77259=CARTESIAN_POINT ( 'NONE',  ( -109.2130836966811387, -284.3900130454696296, -257.3837567132265463 ) ) ;
#77261=CARTESIAN_POINT ( 'NONE',  ( 36.29903743685528639, -282.3616686027557421, -248.9006549765587124 ) ) ;
#77262=CARTESIAN_POINT ( 'NONE',  ( -68.29540153355293342, -273.9673374811358713, -204.2115265979955723 ) ) ;
#77263=CARTESIAN_POINT ( 'NONE',  ( 36.99523792961881696, -286.1145090207178896, -251.8671092167354288 ) ) ;
#77264=CARTESIAN_POINT ( 'NONE',  ( 38.02139949185922774, -282.3102198554902884, -255.7589459090048933 ) ) ;
#77266=CARTESIAN_POINT ( 'NONE',  ( -99.88602327595673103, -279.4891286030614310, -314.0751362733595329 ) ) ;
#77267=CARTESIAN_POINT ( 'NONE',  ( -59.28100680299512248, -280.4268010511798934, -196.6591532262175974 ) ) ;
#77268=CARTESIAN_POINT ( 'NONE',  ( -92.05005921254146983, -276.6952119285918457, -226.6919474004047572 ) ) ;
#77269=CARTESIAN_POINT ( 'NONE',  ( -112.8251851669977412, -274.5109097693414242, -270.3860576588319304 ) ) ;
#77271=CARTESIAN_POINT ( 'NONE',  ( -72.79831222453096018, -275.5819331585354348, -204.4030136627089860 ) ) ;
#77272=CARTESIAN_POINT ( 'NONE',  ( 173.4835934154848474, 243.5194095459789594, -179.5650955095518668 ) ) ;
#77273=CARTESIAN_POINT ( 'NONE',  ( -39.72913769637881387, -278.0421591143949627, -195.7417012399943985 ) ) ;
#77274=CARTESIAN_POINT ( 'NONE',  ( 38.49251824203401640, -295.3830215542195674, -275.9420958396887045 ) ) ;
#77275=CARTESIAN_POINT ( 'NONE',  ( -50.49768193835280528, -294.5731957043777243, -342.2694819639166326 ) ) ;
#77276=CARTESIAN_POINT ( 'NONE',  ( -11.16828578309394437, -291.8918138754450524, -197.9554217367301590 ) ) ;
#77278=CARTESIAN_POINT ( 'NONE',  ( -96.07028261437285721, -294.4641418486955331, -319.2645939763480101 ) ) ;
#77279=CARTESIAN_POINT ( 'NONE',  ( 36.24793321391939571, -286.0330173055198202, -276.5686898780962792 ) ) ;
#77280=CARTESIAN_POINT ( 'NONE',  ( 35.69422701420712940, -295.2392574985910869, -257.0007532810924999 ) ) ;
#77281=CARTESIAN_POINT ( 'NONE',  ( -105.6662596395761682, -285.5059467207601642, -297.5735045685493105 ) ) ;
#77283=CARTESIAN_POINT ( 'NONE',  ( -111.7694017034676790, -291.7299180762429387, -251.5108651682547816 ) ) ;
#77284=CARTESIAN_POINT ( 'NONE',  ( 25.61523959131629624, -282.5544737994703723, -307.5341694113048447 ) ) ;
#77285=CARTESIAN_POINT ( 'NONE',  ( -68.08099987688039789, -294.2418324800765959, -340.5259536945005721 ) ) ;
#77286=CARTESIAN_POINT ( 'NONE',  ( -91.47749177689408384, -290.6016074051137821, -324.9655337851310719 ) ) ;
#77287=CARTESIAN_POINT ( 'NONE',  ( -93.54355141942230034, -290.3266848980300097, -322.9819581056194693 ) ) ;
#77288=CARTESIAN_POINT ( 'NONE',  ( 6.925239249690358534, -286.8402914982984271, -212.2503905482281255 ) ) ;
#77291=CARTESIAN_POINT ( 'NONE',  ( -113.0761406689542099, -298.4576147758664888, -266.8170708179517874 ) ) ;
#77292=CARTESIAN_POINT ( 'NONE',  ( -112.8998493393293785, -295.3892078481714520, -258.2672281377859917 ) ) ;
#77293=CARTESIAN_POINT ( 'NONE',  ( 5.069135742710565218, -279.7002664200090294, -210.6557627097400882 ) ) ;
#77295=CARTESIAN_POINT ( 'NONE',  ( 31.79722804924804080, -275.4949158563856599, -304.2364910928609447 ) ) ;
#77296=CARTESIAN_POINT ( 'NONE',  ( -111.0781455506785989, -295.0177375948194367, -271.4542650046025187 ) ) ;
#77297=CARTESIAN_POINT ( 'NONE',  ( -94.54290868380795132, -279.7527027546158251, -317.6979073773452455 ) ) ;
#77298=CARTESIAN_POINT ( 'NONE',  ( 36.82233284998997647, -273.6363385670197772, -266.0911458571676462 ) ) ;
#77299=CARTESIAN_POINT ( 'NONE',  ( -50.52756109534759332, -296.4293858258642445, -342.5640512630100716 ) ) ;
#77300=CARTESIAN_POINT ( 'NONE',  ( -110.0446187179810238, -297.7604578176957943, -260.5690238123582958 ) ) ;
#77302=CARTESIAN_POINT ( 'NONE',  ( -97.62889640276073067, -297.5236389424904360, -316.9647056497042286 ) ) ;
#77303=CARTESIAN_POINT ( 'NONE',  ( -99.83017026760452950, -271.1403111205165715, -228.1541608417376779 ) ) ;
#77304=CARTESIAN_POINT ( 'NONE',  ( -22.72834790946917494, -292.8955738398317976, -198.7347080154864614 ) ) ;
#77305=CARTESIAN_POINT ( 'NONE',  ( -103.3821449118243265, -288.6904899815788781, -302.8270165252582728 ) ) ;
#77307=CARTESIAN_POINT ( 'NONE',  ( 21.79952980183030675, -275.3820483022533381, -221.1489058207764060 ) ) ;
#77308=CARTESIAN_POINT ( 'NONE',  ( -102.5531277108105570, -297.3326026026563227, -237.3919050365249461 ) ) ;
#77309=CARTESIAN_POINT ( 'NONE',  ( -42.34653686997286570, -281.9692149499761626, -195.1722995795721260 ) ) ;
#77310=CARTESIAN_POINT ( 'NONE',  ( 5.919282313119296646, -279.3103535233535695, -207.2597260016497387 ) ) ;
#77311=CARTESIAN_POINT ( 'NONE',  ( -14.62772986771192407, -276.1140199954659806, -343.8837877214476748 ) ) ;
#77312=CARTESIAN_POINT ( 'NONE',  ( -14.44848591618436195, -278.7438323821601784, -197.6260773797845900 ) ) ;
#77313=CARTESIAN_POINT ( 'NONE',  ( 29.45772765340825217, -281.1517444727174393, -300.3256788491529505 ) ) ;
#77314=CARTESIAN_POINT ( 'NONE',  ( 33.60592920785114046, -279.2294068260043787, -245.3768462868488029 ) ) ;
#77315=CARTESIAN_POINT ( 'NONE',  ( 19.46519033736816340, -273.4692530494965581, -223.5812920476788577 ) ) ;
#77316=CARTESIAN_POINT ( 'NONE',  ( -109.5424002012343152, -280.2906051159577601, -290.7069027285324410 ) ) ;
#77318=DIRECTION ( 'NONE',  ( 0.000000000000000000, 0.000000000000000000, -1.000000000000000000 ) ) ;
#77319=CARTESIAN_POINT ( 'NONE',  ( -15.15586600844804366, -296.5661453759868778, -194.3809848250822085 ) ) ;
#77321=CARTESIAN_POINT ( 'NONE',  ( -8.511219139766771136, -292.4192644703935002, -198.9622148678591600 ) ) ;
#77322=CARTESIAN_POINT ( 'NONE',  ( -35.72478514203644551, -279.0321009713018157, -345.5232069913787996 ) ) ;
#77323=CARTESIAN_POINT ( 'NONE',  ( 28.40162965020363828, -273.0708667732494632, -234.1582794054303065 ) ) ;
#77326=CARTESIAN_POINT ( 'NONE',  ( -110.3366228393558544, -286.7236409346665482, -250.6435797490756272 ) ) ;
#77328=CARTESIAN_POINT ( 'NONE',  ( 29.10142715569293159, -285.0898351751019959, -235.4609823526696175 ) ) ;
#77330=CARTESIAN_POINT ( 'NONE',  ( 34.71126590625547692, -292.5305231445061622, -284.3432705863880301 ) ) ;
#77331=CARTESIAN_POINT ( 'NONE',  ( 18.72437503044040596, -285.0096811931502998, -221.7045593444512690 ) ) ;
#77332=CARTESIAN_POINT ( 'NONE',  ( 27.50960667658514680, -292.0550941587824809, -308.0348309973611549 ) ) ;
#77333=CARTESIAN_POINT ( 'NONE',  ( -91.39805402843452953, -283.7795906197707723, -216.5037289358239150 ) ) ;
#77334=CARTESIAN_POINT ( 'NONE',  ( -110.9580787753649957, -280.2201773017984010, -265.1583102334440127 ) ) ;
#77335=CARTESIAN_POINT ( 'NONE',  ( 36.00963802370197442, -289.0363214940731496, -292.4881452991650121 ) ) ;
#77336=CARTESIAN_POINT ( 'NONE',  ( 37.86509368631639916, -279.9296282722160640, -281.2198553779076633 ) ) ;
#77337=CARTESIAN_POINT ( 'NONE',  ( 24.23834806081161375, -288.0942030010875214, -309.5644043888502210 ) ) ;
#77338=CARTESIAN_POINT ( 'NONE',  ( -95.26581759588367504, -280.6124383379262213, -224.9517165648865102 ) ) ;
#77339=CARTESIAN_POINT ( 'NONE',  ( -6.711125407345084781, -281.2676868631708089, -203.9067202432402155 ) ) ;
#77340=CARTESIAN_POINT ( 'NONE',  ( -66.57476175461849266, -287.6510473258031197, -200.9072850254773925 ) ) ;
#77342=CARTESIAN_POINT ( 'NONE',  ( -18.54997314560486288, -274.2876024936937256, -195.6343329760304073 ) ) ;
#77343=CARTESIAN_POINT ( 'NONE',  ( -100.2138800420910059, -291.9877266598252277, -310.5971192104252623 ) ) ;
#77345=CARTESIAN_POINT ( 'NONE',  ( -37.37352853689063181, -294.5519495502701375, -190.3611179825600175 ) ) ;
#77347=CARTESIAN_POINT ( 'NONE',  ( -75.48002086293303137, -271.5449969381613187, -205.5283310817638665 ) ) ;
#77349=CARTESIAN_POINT ( 'NONE',  ( -107.6449163768319437, -294.5727261290124943, -299.8899149845005923 ) ) ;
#77350=CARTESIAN_POINT ( 'NONE',  ( -70.48986961165952891, -297.1105319472983410, -205.2381535029308282 ) ) ;
#77351=CARTESIAN_POINT ( 'NONE',  ( -69.03882190068929958, -290.9969293095570606, -336.8893091954611236 ) ) ;
#77352=CARTESIAN_POINT ( 'NONE',  ( 27.75682983075313004, -283.7861920194488334, -305.5769582877894095 ) ) ;
#77353=CARTESIAN_POINT ( 'NONE',  ( -31.85085868743179560, -290.4095479473361934, -346.6265049199604960 ) ) ;
#77354=CARTESIAN_POINT ( 'NONE',  ( -41.71551683489051499, -290.4213084805252834, -346.7559810974654511 ) ) ;
#77355=CARTESIAN_POINT ( 'NONE',  ( -11.35217416547049751, -288.3909272591037620, -200.0081138632613715 ) ) ;
#77356=CARTESIAN_POINT ( 'NONE',  ( -48.12088097647951201, -280.0854429653931561, -194.0654917074606089 ) ) ;
#77357=CARTESIAN_POINT ( 'NONE',  ( -81.05885674789219308, -293.7202373202401304, -332.0539615452185558 ) ) ;
#77358=CARTESIAN_POINT ( 'NONE',  ( -69.18839340495958368, -283.2929206411404266, -340.4810822252150615 ) ) ;
#77359=CARTESIAN_POINT ( 'NONE',  ( 25.03493015157739521, -277.9615880738130045, -310.7054365858038523 ) ) ;
#77360=CARTESIAN_POINT ( 'NONE',  ( -54.49178911615187815, -300.3376638359845856, -195.3683826091709363 ) ) ;
#77361=CARTESIAN_POINT ( 'NONE',  ( 21.83750849964845742, -274.4395752303639142, -318.0450448354746982 ) ) ;
#77362=CARTESIAN_POINT ( 'NONE',  ( 133.0872704186301405, -299.5541904835127980, -189.7068768330456123 ) ) ;
#77363=CARTESIAN_POINT ( 'NONE',  ( 35.20010206636703742, -281.1798904496186537, -279.4721262232380354 ) ) ;
#77364=CARTESIAN_POINT ( 'NONE',  ( -112.9049515239061634, -279.5991043119831261, -282.9390254968345175 ) ) ;
#77365=CARTESIAN_POINT ( 'NONE',  ( -85.35638131283359087, -284.4655923995548505, -210.4661215053584726 ) ) ;
#77366=CARTESIAN_POINT ( 'NONE',  ( 22.61257280515301460, -294.7131862893086236, -226.9407363848139312 ) ) ;
#77367=CARTESIAN_POINT ( 'NONE',  ( -13.33405157559051446, -275.9589860885334929, -198.0418727902042804 ) ) ;
#77368=CARTESIAN_POINT ( 'NONE',  ( -96.56505392314146263, -274.5219562103158637, -221.9062537604232830 ) ) ;
#77370=CARTESIAN_POINT ( 'NONE',  ( 3.132342629701405201, -276.3248588337945648, -331.1134995600137358 ) ) ;
#77371=CARTESIAN_POINT ( 'NONE',  ( -97.87682630648174609, -297.9514028538691832, -314.3776039246594678 ) ) ;
#77372=CARTESIAN_POINT ( 'NONE',  ( -110.1432894426382489, -282.7755235744673996, -252.9867443627554167 ) ) ;
#77373=CARTESIAN_POINT ( 'NONE',  ( 38.04206837735083724, -293.0230429012081572, -254.7070203038033185 ) ) ;
#77374=CARTESIAN_POINT ( 'NONE',  ( 23.79889418041276983, -274.1573543743063510, -313.2712431450771078 ) ) ;
#77375=CARTESIAN_POINT ( 'NONE',  ( -26.24076471373900077, -290.5132203334983387, -345.7481834968157273 ) ) ;
#77376=CARTESIAN_POINT ( 'NONE',  ( -109.2446036967447469, -289.2839221563621095, -284.7151912014841173 ) ) ;
#77377=ORIENTED_EDGE ( 'NONE', *, *, #47505, .T. ) ;
#77378=CARTESIAN_POINT ( 'NONE',  ( 28.97333788253397557, -291.6299110244307826, -232.4016392550730927 ) ) ;
#77379=CARTESIAN_POINT ( 'NONE',  ( -104.7209413559483835, -290.5978710534776042, -242.0848330055396787 ) ) ;
#77381=CARTESIAN_POINT ( 'NONE',  ( 37.98397888825627433, -288.4509250956489268, -255.9550570612347826 ) ) ;
#77382=CARTESIAN_POINT ( 'NONE',  ( -92.22713538988517712, -279.5728480591091056, -222.1790755507894062 ) ) ;
#77383=CARTESIAN_POINT ( 'NONE',  ( -65.50283942674079185, -294.3321621436324449, -341.7086054328553928 ) ) ;
#77384=CARTESIAN_POINT ( 'NONE',  ( -113.3878946311204885, -285.3509056830875465, -258.5953143770485667 ) ) ;
#77385=CARTESIAN_POINT ( 'NONE',  ( -83.26666720299689928, -285.7757818577235298, -208.5156694566777560 ) ) ;
#77386=CARTESIAN_POINT ( 'NONE',  ( 35.45046789263039244, -281.9696746804660847, -276.7487675510756162 ) ) ;
#77387=CARTESIAN_POINT ( 'NONE',  ( 103.0508316722241346, 116.5178241089715954, -282.9552863566690348 ) ) ;
#77389=CARTESIAN_POINT ( 'NONE',  ( -23.47725864820640496, -107.6783844017259923, -361.4025868328823776 ) ) ;
#77390=CARTESIAN_POINT ( 'NONE',  ( -98.64580574393880852, -246.0797455245688639, -331.3209657627199931 ) ) ;
#77391=CARTESIAN_POINT ( 'NONE',  ( -6.451524256303274640, -273.6657537687231638, -204.0406930583991993 ) ) ;
#77392=CARTESIAN_POINT ( 'NONE',  ( 15.81258065505600285, -275.1972062376293593, -320.8472399181486026 ) ) ;
#77393=CARTESIAN_POINT ( 'NONE',  ( -65.51362775474740374, -297.2013135087214550, -198.7089991478085551 ) ) ;
#77394=CARTESIAN_POINT ( 'NONE',  ( -46.28360890110539572, -155.9045745473734712, -362.0530608825127956 ) ) ;
#77395=CARTESIAN_POINT ( 'NONE',  ( 3.225720779939448946, -275.2044512057388488, -335.2893538922770631 ) ) ;
#77396=CARTESIAN_POINT ( 'NONE',  ( -32.64886520893520583, -275.8722196026442361, -196.4840060102316670 ) ) ;
#77398=CARTESIAN_POINT ( 'NONE',  ( -112.0481483480647711, -297.7149128191339855, -252.7041984195134035 ) ) ;
#77400=CARTESIAN_POINT ( 'NONE',  ( -26.45953640725284473, -289.4024252463407834, -342.6587813542579966 ) ) ;
#77401=CARTESIAN_POINT ( 'NONE',  ( -92.57381523852140504, -296.6216133328625801, -323.7799562400920763 ) ) ;
#77402=CARTESIAN_POINT ( 'NONE',  ( -113.8813637145674420, -296.9465763628708714, -278.1845955469045748 ) ) ;
#77403=CARTESIAN_POINT ( 'NONE',  ( -3.638144592954465129, -292.6767044796009145, -205.6071964888223249 ) ) ;
#77405=CARTESIAN_POINT ( 'NONE',  ( 35.85008965298685268, -277.7116598873871567, -289.1301379266436697 ) ) ;
#77407=CARTESIAN_POINT ( 'NONE',  ( 37.27310987508800366, -280.8248233538912473, -251.5952705020294502 ) ) ;
#77408=CARTESIAN_POINT ( 'NONE',  ( -74.12110925451041510, -278.4951698956776909, -333.6910754478980152 ) ) ;
#77409=CARTESIAN_POINT ( 'NONE',  ( 15.30855924699483595, -276.5438962422526288, -215.5712995857689407 ) ) ;
#77410=CARTESIAN_POINT ( 'NONE',  ( -104.8825883084782902, -276.1320843338635882, -303.8946880390452066 ) ) ;
#77411=CARTESIAN_POINT ( 'NONE',  ( -109.8384292365054478, -297.3322686944680981, -260.5913291757692036 ) ) ;
#77412=CARTESIAN_POINT ( 'NONE',  ( -80.51501540564287041, -294.2252114374209100, -329.9550754243879851 ) ) ;
#77414=CARTESIAN_POINT ( 'NONE',  ( 6.144306111678071503, -281.1175836400039429, -206.8906983809304450 ) ) ;
#77415=CARTESIAN_POINT ( 'NONE',  ( -13.78339066984367811, -276.9045424514074512, -339.5084388980351946 ) ) ;
#77416=CARTESIAN_POINT ( 'NONE',  ( 39.20877648171386198, -286.2520745157656847, -271.5603816381632214 ) ) ;
#77417=CARTESIAN_POINT ( 'NONE',  ( -111.5687934622130797, -274.6947677400971202, -259.2664601885816751 ) ) ;
#77418=CARTESIAN_POINT ( 'NONE',  ( 82.66796173774982037, -298.0572237680152057, -197.3908676648706546 ) ) ;
#77419=CARTESIAN_POINT ( 'NONE',  ( -8.163471781230724034, -287.8572653847649576, -337.5064996368687389 ) ) ;
#77421=CARTESIAN_POINT ( 'NONE',  ( -35.61702189677296104, -278.3139081398977055, -196.3553038020013162 ) ) ;
#77422=CARTESIAN_POINT ( 'NONE',  ( -34.27071471297013261, -278.6662055073705915, -196.8233486303982431 ) ) ;
#77423=CARTESIAN_POINT ( 'NONE',  ( -83.71043491836863382, -281.7735895281192029, -328.6617593302388514 ) ) ;
#77424=CARTESIAN_POINT ( 'NONE',  ( 17.95762232805615000, -288.8445455696343060, -219.6769646416762782 ) ) ;
#77425=CARTESIAN_POINT ( 'NONE',  ( -95.57876355041473460, -279.1321192728485698, -315.0329765732262217 ) ) ;
#77427=CARTESIAN_POINT ( 'NONE',  ( -67.54727592993694429, -293.6560919845480271, -201.6985686519389276 ) ) ;
#77428=CARTESIAN_POINT ( 'NONE',  ( -37.15229770530419984, -275.2896422888138659, -346.3604383442195740 ) ) ;
#77429=CARTESIAN_POINT ( 'NONE',  ( 5.463179849941725230, -277.1070847272241053, -329.6826813774569587 ) ) ;
#77430=CARTESIAN_POINT ( 'NONE',  ( 8.120700661274417698, -284.4322384300798490, -330.2209420551196786 ) ) ;
#77431=DIRECTION ( 'NONE',  ( -1.000000000000000000, -0.000000000000000000, -0.000000000000000000 ) ) ;
#77432=CARTESIAN_POINT ( 'NONE',  ( -97.86082782334997887, -291.8586552450849467, -315.6235199801517979 ) ) ;
#77433=CARTESIAN_POINT ( 'NONE',  ( -106.5383782189670541, -294.1727330861852465, -299.4213802197311907 ) ) ;
#77434=CARTESIAN_POINT ( 'NONE',  ( -91.78136191330990812, -284.4967643776529940, -216.1349061936205658 ) ) ;
#77436=CARTESIAN_POINT ( 'NONE',  ( -21.81361185470477437, -272.9401739851583670, -198.5271291531404358 ) ) ;
#77437=CARTESIAN_POINT ( 'NONE',  ( 34.63802555264857830, -291.9274201760563301, -288.5210897342315093 ) ) ;
#77440=CARTESIAN_POINT ( 'NONE',  ( -86.05540008278258313, -289.8712145154160567, -211.5585211824224245 ) ) ;
#77441=CARTESIAN_POINT ( 'NONE',  ( -26.74001617445735590, -284.4249468900777060, -195.0648615902831011 ) ) ;
#77443=CARTESIAN_POINT ( 'NONE',  ( -102.2827404765905470, -285.5082187710081030, -305.0821826743190286 ) ) ;
#77444=CARTESIAN_POINT ( 'NONE',  ( -25.12489836091869932, -287.0146202568702734, -198.1754472287298086 ) ) ;
#77445=CARTESIAN_POINT ( 'NONE',  ( -101.8217727014944671, -293.0532480950006970, -231.2639581509192510 ) ) ;
#77446=CARTESIAN_POINT ( 'NONE',  ( 24.86715268174845050, -274.2100772408344938, -313.3395480074868260 ) ) ;
#77448=CARTESIAN_POINT ( 'NONE',  ( 34.70047193010576336, -275.5421872205032514, -243.2378855682353560 ) ) ;
#77449=CARTESIAN_POINT ( 'NONE',  ( -36.37181904703815150, -290.1440745006411248, -194.7945497292644177 ) ) ;
#77450=CARTESIAN_POINT ( 'NONE',  ( -111.4405165336055887, -278.2897470859475106, -291.2982956171031219 ) ) ;
#77451=CARTESIAN_POINT ( 'NONE',  ( -112.0294948340390278, -298.5171885865095760, -271.5131086094469879 ) ) ;
#77454=CARTESIAN_POINT ( 'NONE',  ( -100.0212152562736065, -283.7633581369656213, -231.8907389205920140 ) ) ;
#77455=CARTESIAN_POINT ( 'NONE',  ( -17.49604334400470051, -278.3080528014002084, -198.0344247584943957 ) ) ;
#77457=CARTESIAN_POINT ( 'NONE',  ( -13.26275721310359756, -272.8392384892069913, -197.9531608251776618 ) ) ;
#77459=CARTESIAN_POINT ( 'NONE',  ( -104.3681639590162575, -277.5074553877019525, -299.6658236221556990 ) ) ;
#77461=CARTESIAN_POINT ( 'NONE',  ( 30.13257583076671864, -295.4671337331292875, -299.9909987527423709 ) ) ;
#77462=CARTESIAN_POINT ( 'NONE',  ( 14.96061581304658716, -279.6891171697345158, -214.1996500705374444 ) ) ;
#77463=CARTESIAN_POINT ( 'NONE',  ( -92.35954251701267026, -296.8055902883151589, -318.6979100505135420 ) ) ;
#77464=CARTESIAN_POINT ( 'NONE',  ( -76.81335628257380677, -296.8837969734492503, -335.9611801973882734 ) ) ;
#77465=CARTESIAN_POINT ( 'NONE',  ( -107.2155191820545355, -272.5016592212732576, -248.9809439852922708 ) ) ;
#77466=CARTESIAN_POINT ( 'NONE',  ( -112.3691769910507219, -292.5770464865422582, -268.4351378432108959 ) ) ;
#77467=CARTESIAN_POINT ( 'NONE',  ( -54.96667055546318892, -285.9982447090957862, -195.4053949060794935 ) ) ;
#77468=CARTESIAN_POINT ( 'NONE',  ( 31.44179341029144226, -273.2772771883630867, -238.4691902126157004 ) ) ;
#77469=CARTESIAN_POINT ( 'NONE',  ( -65.44900140514982922, -289.2428097963760365, -342.1041383990375380 ) ) ;
#77470=CARTESIAN_POINT ( 'NONE',  ( -75.36486859066312149, -281.5228309509111000, -206.0670845502641271 ) ) ;
#77471=CARTESIAN_POINT ( 'NONE',  ( -38.61702128718089710, -285.0945527850954022, -197.1244058867658850 ) ) ;
#77472=CARTESIAN_POINT ( 'NONE',  ( -109.6964322990371414, -288.8064335137029275, -250.5692621599298491 ) ) ;
#77473=CARTESIAN_POINT ( 'NONE',  ( 22.29632774050155319, -23.10002859818378340, -338.8215327972035311 ) ) ;
#77474=CARTESIAN_POINT ( 'NONE',  ( 31.90091445477538556, -286.7503814197424390, -247.0491303502828373 ) ) ;
#77476=CARTESIAN_POINT ( 'NONE',  ( 38.19619376431163715, -282.6657930535725995, -284.1033839688629996 ) ) ;
#77477=CARTESIAN_POINT ( 'NONE',  ( -112.0365359206662390, -289.3880832818108502, -288.1233777822968705 ) ) ;
#77478=CARTESIAN_POINT ( 'NONE',  ( -111.0483736974109519, -279.9071461720388925, -289.7453811506374564 ) ) ;
#77479=CARTESIAN_POINT ( 'NONE',  ( -69.76869561916049634, -280.9492800978976561, -201.0518830684958402 ) ) ;
#77480=CARTESIAN_POINT ( 'NONE',  ( 33.93995540664759147, -281.5931829933286394, -286.1067709943074533 ) ) ;
#77481=CARTESIAN_POINT ( 'NONE',  ( 37.36812384980096624, -277.4604354034465246, -263.2052621739371716 ) ) ;
#77482=CARTESIAN_POINT ( 'NONE',  ( -72.07403543291064807, -295.4987540259543835, -339.0827658402249654 ) ) ;
#77483=CARTESIAN_POINT ( 'NONE',  ( -87.00497514474724881, -289.3772740435469473, -214.5653989026564261 ) ) ;
#77484=CARTESIAN_POINT ( 'NONE',  ( -47.30119167050533235, -296.8430903940855501, -197.6802581844369229 ) ) ;
#77487=CARTESIAN_POINT ( 'NONE',  ( 33.61117802323219195, -283.7670275350053544, -293.0459090269075659 ) ) ;
#77488=CARTESIAN_POINT ( 'NONE',  ( -93.10128784045257078, -295.5488107609818371, -317.5287228185309232 ) ) ;
#77489=CARTESIAN_POINT ( 'NONE',  ( 33.03526250480244641, -294.2419330457668707, -239.8885788777388086 ) ) ;
#77490=CARTESIAN_POINT ( 'NONE',  ( -37.53246934173292715, -283.7060525861120936, -343.4752490306422033 ) ) ;
#77491=CARTESIAN_POINT ( 'NONE',  ( -15.83176370678345712, -273.3824027561016692, -196.6164422370010527 ) ) ;
#77492=CARTESIAN_POINT ( 'NONE',  ( -39.21753122765307609, -292.6806326328924115, -193.4729152999338169 ) ) ;
#77493=CARTESIAN_POINT ( 'NONE',  ( -21.22327490183170084, -284.3963737000675565, -196.3307063532376162 ) ) ;
#77494=CARTESIAN_POINT ( 'NONE',  ( -112.5437777050342874, -290.6797251057994913, -286.8047130811607985 ) ) ;
#77495=CARTESIAN_POINT ( 'NONE',  ( 7.996389700461218553, -288.7457765152440174, -327.6022316804633761 ) ) ;
#77498=CARTESIAN_POINT ( 'NONE',  ( -109.7947985209783184, -268.5820228192868058, -295.2857659021627228 ) ) ;
#77499=CARTESIAN_POINT ( 'NONE',  ( -49.95962354570519182, -284.7303189076574199, -345.6707071636948285 ) ) ;
#77500=CARTESIAN_POINT ( 'NONE',  ( -110.4542110544635705, -282.2666405000204009, -253.6410175316879361 ) ) ;
#77502=CARTESIAN_POINT ( 'NONE',  ( 31.64081303228361008, -280.8033101443431860, -295.3232035731341512 ) ) ;
#77503=CARTESIAN_POINT ( 'NONE',  ( 23.49872483143495572, -275.8490079095890906, -317.5437816025196298 ) ) ;
#77504=CARTESIAN_POINT ( 'NONE',  ( -43.93743976431574083, -281.9688793267448546, -195.7675226082509141 ) ) ;
#77505=CARTESIAN_POINT ( 'NONE',  ( -75.44914023181735274, -209.3092839176353834, -355.0955389360644290 ) ) ;
#77506=CARTESIAN_POINT ( 'NONE',  ( 36.42100054318044045, -279.8746630386589231, -250.3697823562115445 ) ) ;
#77507=CARTESIAN_POINT ( 'NONE',  ( -44.14984519467542867, -283.9857342012782624, -196.0274381112338631 ) ) ;
#77508=CARTESIAN_POINT ( 'NONE',  ( -112.6452589435766214, -298.1785821128481189, -280.9116697671348675 ) ) ;
#77509=CARTESIAN_POINT ( 'NONE',  ( 16.77954800854531570, -293.3411276293782066, -221.2065927208255971 ) ) ;
#77511=CARTESIAN_POINT ( 'NONE',  ( -66.74610779413268347, -290.3434458811649392, -203.0066505072790051 ) ) ;
#77512=CARTESIAN_POINT ( 'NONE',  ( -4.031487858280806691, -277.2757704414927389, -339.6846350234554279 ) ) ;
#77513=CARTESIAN_POINT ( 'NONE',  ( -57.90681300412333599, -297.9456681201089054, -200.3177304510961108 ) ) ;
#77515=CARTESIAN_POINT ( 'NONE',  ( -71.25369382832650444, -272.5352302795299124, -201.5754421881898395 ) ) ;
#77520=CARTESIAN_POINT ( 'NONE',  ( 22.84638299952234775, -283.2126858954650288, -312.2134861756413784 ) ) ;
#77521=CARTESIAN_POINT ( 'NONE',  ( 10.86723799987209915, -284.1564117300929411, -329.1648366521967546 ) ) ;
#77522=CARTESIAN_POINT ( 'NONE',  ( -95.31001273124209661, -282.9825817881678063, -315.1374100938461993 ) ) ;
#77523=CARTESIAN_POINT ( 'NONE',  ( 26.18118139920536791, -282.8913964389785178, -231.8465947934172675 ) ) ;
#77524=CARTESIAN_POINT ( 'NONE',  ( 35.79168975985043488, -274.1558180669345575, -279.8344837313644575 ) ) ;
#77527=CARTESIAN_POINT ( 'NONE',  ( 25.53390351464331687, -276.1143329836826297, -232.5682004054660297 ) ) ;
#77530=CARTESIAN_POINT ( 'NONE',  ( -56.87309220113347408, -278.1005115891152286, -344.7308129160258545 ) ) ;
#77534=CARTESIAN_POINT ( 'NONE',  ( -111.1616828378459729, -286.6293528005825806, -253.3048687552398235 ) ) ;
#77535=CARTESIAN_POINT ( 'NONE',  ( -82.46742585626191158, -294.8834249094667825, -328.0127857633279973 ) ) ;
#77536=CARTESIAN_POINT ( 'NONE',  ( 3.119437538161993206, -287.8728050301662051, -335.8163091276400678 ) ) ;
#77538=CARTESIAN_POINT ( 'NONE',  ( -94.89608127450399877, -283.4413473251815390, -223.8064584945653905 ) ) ;
#77539=CARTESIAN_POINT ( 'NONE',  ( -104.6595739868808437, -282.7300381500899107, -300.0878529975846618 ) ) ;
#77540=CARTESIAN_POINT ( 'NONE',  ( -2.914725045224477284, -286.8308839122032055, -335.9370060928645216 ) ) ;
#77541=CARTESIAN_POINT ( 'NONE',  ( -110.2654406331460706, -285.6423026439239834, -279.1208975253079529 ) ) ;
#77542=CARTESIAN_POINT ( 'NONE',  ( 11.38540089847801084, -274.3764101281125818, -327.3757676031328288 ) ) ;
#77543=CARTESIAN_POINT ( 'NONE',  ( -10.25903341187131979, -284.7995405243312348, -199.0801187794445184 ) ) ;
#77544=CARTESIAN_POINT ( 'NONE',  ( -21.07843767550062708, -300.2558935330509371, -195.3555647147243519 ) ) ;
#77545=CARTESIAN_POINT ( 'NONE',  ( -21.34860693657575581, -284.2566516374712364, -196.9155640420842417 ) ) ;
#77546=CARTESIAN_POINT ( 'NONE',  ( -39.72084680147518299, -280.9628309990401362, -197.1519179504336421 ) ) ;
#77547=CARTESIAN_POINT ( 'NONE',  ( 37.27397641609041301, -289.6740782640075054, -279.8654853146505275 ) ) ;
#77549=DIRECTION ( 'NONE',  ( 1.000000000000000000, 0.000000000000000000, 0.000000000000000000 ) ) ;
#77550=CARTESIAN_POINT ( 'NONE',  ( -66.34859727899481641, -297.3490992430853908, -340.1454904656250164 ) ) ;
#77553=CARTESIAN_POINT ( 'NONE',  ( -11.01795387066295184, -278.3949851673045259, -200.0775535118540347 ) ) ;
#77554=CARTESIAN_POINT ( 'NONE',  ( -111.8354981165519604, -289.9861155769526704, -251.4711408001130621 ) ) ;
#77555=CARTESIAN_POINT ( 'NONE',  ( -70.09726791484126807, -293.8910117257324259, -336.4936606259843757 ) ) ;
#77556=CARTESIAN_POINT ( 'NONE',  ( -49.20513046525081791, -278.5826102365383576, -197.8317963427482766 ) ) ;
#77557=CARTESIAN_POINT ( 'NONE',  ( -35.75929806470490746, -296.2117496729896402, -196.1264183674259982 ) ) ;
#77558=CARTESIAN_POINT ( 'NONE',  ( 33.22837610134417474, -295.1374886194453779, -290.9272985017212818 ) ) ;
#77559=CARTESIAN_POINT ( 'NONE',  ( -54.42813229853332757, -291.7662352645559167, -345.3683826091709648 ) ) ;
#77560=CARTESIAN_POINT ( 'NONE',  ( -111.5951682169763473, -295.2539372854956241, -252.7790182125252443 ) ) ;
#77561=CARTESIAN_POINT ( 'NONE',  ( -3.748867461086582420, -290.7291090862343026, -202.1888963750468236 ) ) ;
#77563=CARTESIAN_POINT ( 'NONE',  ( -108.6841585681019922, -292.2142887924738375, -252.2646370473189847 ) ) ;
#77565=CARTESIAN_POINT ( 'NONE',  ( -30.80269962062244815, -292.9397581282994452, -197.4924470784148980 ) ) ;
#77566=CARTESIAN_POINT ( 'NONE',  ( -105.6569842320517552, -292.2070231878549862, -235.5882255541883978 ) ) ;
#77567=CARTESIAN_POINT ( 'NONE',  ( 35.02731207708480099, -279.3025990722478582, -249.3116408422868062 ) ) ;
#77568=CARTESIAN_POINT ( 'NONE',  ( 8.848840249748281650, -292.7059267529546105, -213.7673825572400688 ) ) ;
#77569=CARTESIAN_POINT ( 'NONE',  ( -38.16990651973561910, -280.0420416017230423, -193.3655721752028853 ) ) ;
#77570=CARTESIAN_POINT ( 'NONE',  ( -38.73642072112740919, -282.7359182163079367, -347.3273381450512716 ) ) ;
#77571=CARTESIAN_POINT ( 'NONE',  ( -95.54590254773420099, -287.9030632454436045, -317.3962033094007325 ) ) ;
#77572=CARTESIAN_POINT ( 'NONE',  ( -13.14883539007644941, -280.8742238869150469, -340.5980335969160819 ) ) ;
#77573=CARTESIAN_POINT ( 'NONE',  ( -77.11446277149565276, -278.0096369106523184, -205.1782616642073265 ) ) ;
#77574=CARTESIAN_POINT ( 'NONE',  ( 24.46235161041294504, -285.8669373949409191, -224.9546019395624796 ) ) ;
#77576=CARTESIAN_POINT ( 'NONE',  ( 25.51871704263546192, -294.6238995836630465, -231.5988065330656411 ) ) ;
#77577=CARTESIAN_POINT ( 'NONE',  ( 37.36543594177911842, -276.7744240220985716, -254.2540778325939073 ) ) ;
#77578=CARTESIAN_POINT ( 'NONE',  ( -109.9255271171182500, -278.1077361699048538, -278.7880431935706724 ) ) ;
#77579=CARTESIAN_POINT ( 'NONE',  ( -111.6333564419386022, -290.9729238740556525, -250.0688033837156752 ) ) ;
#77581=CARTESIAN_POINT ( 'NONE',  ( -33.16328871464007477, -281.0797917528433914, -345.8183914831684547 ) ) ;
#77582=CARTESIAN_POINT ( 'NONE',  ( 2.378148933008505939, -291.6571635687413959, -208.7726550309245397 ) ) ;
#77583=CARTESIAN_POINT ( 'NONE',  ( -107.5739001937540564, -294.2085732501393522, -296.8220079075608737 ) ) ;
#77587=CARTESIAN_POINT ( 'NONE',  ( -75.00596157585009394, -291.0437860298532655, -207.6970091394162523 ) ) ;
#77589=CARTESIAN_POINT ( 'NONE',  ( -102.0172624299486870, -298.6233781216987495, -301.5434626090942061 ) ) ;
#77590=CARTESIAN_POINT ( 'NONE',  ( -113.8851927030090252, -295.6922264361884345, -263.8783595288938386 ) ) ;
#77591=CARTESIAN_POINT ( 'NONE',  ( 18.26988535788170154, -278.9794544989266569, -218.9057291438649884 ) ) ;
#77593=CARTESIAN_POINT ( 'NONE',  ( -87.98249520661562428, -285.0579179958273812, -327.7799726252342225 ) ) ;
#77594=CARTESIAN_POINT ( 'NONE',  ( -9.491425486574028625, -286.2598194801654472, -202.8690043349675420 ) ) ;
#77596=CARTESIAN_POINT ( 'NONE',  ( -94.12803802724369007, -279.4124638351806880, -317.3491652886649490 ) ) ;
#77597=CARTESIAN_POINT ( 'NONE',  ( -109.0322021264194632, -294.8412171737081167, -249.5688423183820817 ) ) ;
#77598=CARTESIAN_POINT ( 'NONE',  ( -111.2251547171315309, -298.3693256925972719, -265.9782936212701543 ) ) ;
#77599=CARTESIAN_POINT ( 'NONE',  ( -73.04852903633221217, -276.3315117055853989, -334.5016495862799388 ) ) ;
#77602=CARTESIAN_POINT ( 'NONE',  ( -114.2129711458231611, -296.1566646993842369, -275.3337762793937600 ) ) ;
#77603=CARTESIAN_POINT ( 'NONE',  ( -104.1267933230056997, -292.0353779681522042, -303.2406788346667668 ) ) ;
#77604=CARTESIAN_POINT ( 'NONE',  ( -112.7724044462825219, -274.5149434905746944, -270.3861090177667847 ) ) ;
#77607=CARTESIAN_POINT ( 'NONE',  ( 1.266038376184138503, -279.6129928427387767, -203.9510439291099146 ) ) ;
#77608=CARTESIAN_POINT ( 'NONE',  ( -113.8409726979541858, -297.1056167466742863, -278.1825042208197374 ) ) ;
#77609=CARTESIAN_POINT ( 'NONE',  ( -81.19583560464567995, -289.6026993450278724, -208.5782702029881364 ) ) ;
#77610=CARTESIAN_POINT ( 'NONE',  ( -40.44365699919875112, -298.3475708375403315, -193.3926738376565879 ) ) ;
#77611=CARTESIAN_POINT ( 'NONE',  ( 24.86365848257481304, -293.3572564928084034, -232.0214321816955874 ) ) ;
#77616=CARTESIAN_POINT ( 'NONE',  ( -54.32826532151603516, -290.7864940015391539, -344.8072986019737414 ) ) ;
#77617=CARTESIAN_POINT ( 'NONE',  ( -37.30987171927208124, -279.5519495502701375, -350.3611179825600175 ) ) ;
#77619=CARTESIAN_POINT ( 'NONE',  ( 38.56588731261480518, -281.0558342886508285, -282.7457948011403914 ) ) ;
#77620=CARTESIAN_POINT ( 'NONE',  ( -111.9208386496081573, -286.4730103291483374, -276.5239518980328057 ) ) ;
#77621=CARTESIAN_POINT ( 'NONE',  ( 37.45053337412381467, -285.9289307630767212, -254.6539061944536684 ) ) ;
#77622=CARTESIAN_POINT ( 'NONE',  ( -86.49567292929069140, -271.3678742391825267, -213.8658793018547328 ) ) ;
#77623=CARTESIAN_POINT ( 'NONE',  ( -94.90724018450953281, -275.1280904704206023, -223.1445398048015534 ) ) ;
#77624=CARTESIAN_POINT ( 'NONE',  ( -110.6914914859981849, -288.8000041624377445, -257.3739644369967436 ) ) ;
#77625=CARTESIAN_POINT ( 'NONE',  ( -103.8793326444933172, -279.9359788209610542, -306.5971351089248742 ) ) ;
#77626=CARTESIAN_POINT ( 'NONE',  ( -110.1683457724123230, -278.4767253480942486, -276.0788831266825696 ) ) ;
#77627=CARTESIAN_POINT ( 'NONE',  ( -32.94861105629794196, -279.4575439087968221, -197.3913061646499045 ) ) ;
#77628=CARTESIAN_POINT ( 'NONE',  ( -17.42487434981083894, -277.8806484263906214, -344.4206383687808852 ) ) ;
#77629=CARTESIAN_POINT ( 'NONE',  ( -81.99489083885298157, -278.2532004084110895, -208.1188391287203387 ) ) ;
#77630=CARTESIAN_POINT ( 'NONE',  ( -72.06482525295078290, -195.1395164891845297, -357.9071827626919458 ) ) ;
#77631=CARTESIAN_POINT ( 'NONE',  ( 98.82013943189359395, -300.5191071293656364, -193.5044647189510840 ) ) ;
#77634=CARTESIAN_POINT ( 'NONE',  ( 97.87027569496429180, -301.1390480024426779, -193.9182337029051837 ) ) ;
#77635=CARTESIAN_POINT ( 'NONE',  ( 39.58706461736021254, -290.0519495502703080, -270.3284710469133074 ) ) ;
#77638=CARTESIAN_POINT ( 'NONE',  ( 34.00799630816176489, -288.4099563119616505, -253.4710270386866284 ) ) ;
#77639=CARTESIAN_POINT ( 'NONE',  ( 36.38808773228214477, -289.0792462829769534, -251.9792682727587305 ) ) ;
#77640=CARTESIAN_POINT ( 'NONE',  ( -37.27624396484597469, -288.3998967430293874, -343.4630220896499395 ) ) ;
#77641=CARTESIAN_POINT ( 'NONE',  ( -99.29095730970597344, -284.6674710412652871, -224.6465403266671785 ) ) ;
#77642=CARTESIAN_POINT ( 'NONE',  ( 21.16247624817584949, -279.3255753297187880, -225.3549980517821041 ) ) ;
#77643=CARTESIAN_POINT ( 'NONE',  ( -9.044108566336742427, -288.2865880865172130, -201.7171295329684426 ) ) ;
#77644=CARTESIAN_POINT ( 'NONE',  ( 30.66873245133542625, -279.6549542470181109, -241.9835068926161057 ) ) ;
#77645=CARTESIAN_POINT ( 'NONE',  ( -95.18933739385968806, -280.5023578947685223, -225.0099136557651889 ) ) ;
#77646=CARTESIAN_POINT ( 'NONE',  ( -89.12501638499873025, -278.2968334431417361, -321.9739716885067651 ) ) ;
#77647=CARTESIAN_POINT ( 'NONE',  ( 2.958121926282671232, -287.3192317577753556, -335.5688122964978106 ) ) ;
#77648=CARTESIAN_POINT ( 'NONE',  ( 0.7971106087138253304, -283.3597769747145776, -337.0815659215375604 ) ) ;
#77649=CARTESIAN_POINT ( 'NONE',  ( -92.38532991824372687, -284.3064911333286204, -324.1172871420218939 ) ) ;
#77650=CARTESIAN_POINT ( 'NONE',  ( 11.91825224058169752, -282.5110361062631910, -324.2355747976889120 ) ) ;
#77651=ORIENTED_EDGE ( 'NONE', *, *, #80097, .F. ) ;
#77654=CARTESIAN_POINT ( 'NONE',  ( -111.3535624238246271, -292.2066126722993999, -286.5645041727724447 ) ) ;
#77656=CARTESIAN_POINT ( 'NONE',  ( 17.15020131634659251, -291.4940543938898827, -216.5842576658749294 ) ) ;
#77657=CARTESIAN_POINT ( 'NONE',  ( -13.97907046121468966, -273.4215907156046228, -200.9522137781057438 ) ) ;
#77658=CARTESIAN_POINT ( 'NONE',  ( 23.94271087561843459, -293.5204018280648484, -316.8103779863600380 ) ) ;
#77659=CARTESIAN_POINT ( 'NONE',  ( -103.4760910022184675, -288.5956555767142504, -302.8718868784371239 ) ) ;
#77660=CARTESIAN_POINT ( 'NONE',  ( 35.71778792059226504, -291.6368684180904438, -258.4375140722710853 ) ) ;
#77661=CARTESIAN_POINT ( 'NONE',  ( -109.0473625289618695, -291.5509763127051883, -286.0856443043307991 ) ) ;
#77663=CARTESIAN_POINT ( 'NONE',  ( -104.2322080542952705, -293.0019800083869654, -236.3251439875608924 ) ) ;
#77664=CARTESIAN_POINT ( 'NONE',  ( -110.5263150196137332, -288.7716880657255274, -253.2135066475688632 ) ) ;
#77665=CARTESIAN_POINT ( 'NONE',  ( -29.01272374781387953, -294.1577551507367616, -195.7734868572562732 ) ) ;
#77666=CARTESIAN_POINT ( 'NONE',  ( 20.51920604996066899, -287.8630761712044546, -225.4665305011370720 ) ) ;
#77667=CARTESIAN_POINT ( 'NONE',  ( 10.06234116798146516, -296.4011405614946284, -328.7624660474543248 ) ) ;
#77669=CARTESIAN_POINT ( 'NONE',  ( 3.940544494944215437, -276.5845743567022623, -207.2580977677613419 ) ) ;
#77670=CARTESIAN_POINT ( 'NONE',  ( -102.1746539962912124, -296.2910279576142898, -229.1197926763808539 ) ) ;
#77671=CARTESIAN_POINT ( 'NONE',  ( 33.47958729538950706, -274.0733400833900646, -291.9066178841515011 ) ) ;
#77672=CARTESIAN_POINT ( 'NONE',  ( 14.35235124876298052, -278.8650816931276495, -216.7258482153007151 ) ) ;
#77673=CARTESIAN_POINT ( 'NONE',  ( -94.93377901851911815, -274.3958067380647208, -224.8607558379044633 ) ) ;
#77674=CARTESIAN_POINT ( 'NONE',  ( -1.561216526088839540, -273.0917775835797556, -202.8454658172614984 ) ) ;
#77676=CARTESIAN_POINT ( 'NONE',  ( -109.1630091193064231, -297.7676108451970549, -286.3946607564227520 ) ) ;
#77678=CARTESIAN_POINT ( 'NONE',  ( -102.9083441053576990, -296.9145749786466126, -302.9350358127435356 ) ) ;
#77680=CARTESIAN_POINT ( 'NONE',  ( 28.70241879707406696, -285.0908619848139551, -233.9680596373990795 ) ) ;
#77681=CARTESIAN_POINT ( 'NONE',  ( -108.5344255438734393, -272.5984244505103220, -254.2181364607774583 ) ) ;
#77682=CIRCLE ( 'NONE', #14238, 3.491568894204821749 ) ;
#77683=CARTESIAN_POINT ( 'NONE',  ( 5.179676330621761693, -286.6097201150020055, -206.1031211403636974 ) ) ;
#77684=CARTESIAN_POINT ( 'NONE',  ( -70.63376909783086433, -289.1458729638741829, -339.7829659757355785 ) ) ;
#77685=CARTESIAN_POINT ( 'NONE',  ( -74.98069705552798325, -299.5337533976257873, -205.0194274155513483 ) ) ;
#77686=CARTESIAN_POINT ( 'NONE',  ( -69.32342310327962309, -293.4736863280037369, -338.0301870168362939 ) ) ;
#77687=CARTESIAN_POINT ( 'NONE',  ( 34.17788284581840941, -280.3908214287328633, -242.1247786582720494 ) ) ;
#77688=CARTESIAN_POINT ( 'NONE',  ( -95.95921662488163406, -288.6952119285919025, -223.5744983911110353 ) ) ;
#77691=CARTESIAN_POINT ( 'NONE',  ( 18.11552068165402218, -287.0292726596195507, -318.5165774165824359 ) ) ;
#77694=CARTESIAN_POINT ( 'NONE',  ( -74.55896841310922696, -287.5470648371380094, -335.4902537927671347 ) ) ;
#77695=CARTESIAN_POINT ( 'NONE',  ( -109.2153664135543920, -274.2849532673811268, -254.0858653124740272 ) ) ;
#77696=CARTESIAN_POINT ( 'NONE',  ( -6.485081694435876898, -281.8747592092881291, -200.4436278864384633 ) ) ;
#77697=CARTESIAN_POINT ( 'NONE',  ( -102.9665184239086955, -271.1289390746248387, -232.8035707031289405 ) ) ;
#77698=CARTESIAN_POINT ( 'NONE',  ( 33.11358151885879408, -281.2991890548242964, -251.2069255579692992 ) ) ;
#77699=CARTESIAN_POINT ( 'NONE',  ( -88.60384951804989839, -295.9143477658249708, -327.8886170038253454 ) ) ;
#77700=CARTESIAN_POINT ( 'NONE',  ( -108.5146180578946087, -274.2247276866234529, -251.4628462230623143 ) ) ;
#77702=CARTESIAN_POINT ( 'NONE',  ( 35.60913324842847061, -283.7765328666387745, -287.8279445386277189 ) ) ;
#77703=CARTESIAN_POINT ( 'NONE',  ( -35.12682494449100545, -297.1392939730989724, -197.1261868491516793 ) ) ;
#77706=CARTESIAN_POINT ( 'NONE',  ( -109.6811386451170733, -286.2944316258024173, -288.7690630320087735 ) ) ;
#77708=CARTESIAN_POINT ( 'NONE',  ( -55.63300648810263738, -274.7666405000204009, -350.3538533559490702 ) ) ;
#77709=CARTESIAN_POINT ( 'NONE',  ( 10.41767779954267148, -275.6093752139835260, -330.6220813604535920 ) ) ;
#77710=CARTESIAN_POINT ( 'NONE',  ( -71.71528547095849149, -285.0352177387784991, -335.5467328413386099 ) ) ;
#77711=CARTESIAN_POINT ( 'NONE',  ( 28.75598869072684849, -277.5939111845766547, -303.3022290863825674 ) ) ;
#77712=CARTESIAN_POINT ( 'NONE',  ( -65.02168542937295115, -284.8320352078922610, -341.5961685025373527 ) ) ;
#77713=CARTESIAN_POINT ( 'NONE',  ( -85.13187999667241002, -282.5244508506763736, -326.0677532411175434 ) ) ;
#77714=CARTESIAN_POINT ( 'NONE',  ( -1.019187615599564056, -282.5344932064879799, -204.7434699374900617 ) ) ;
#77715=CARTESIAN_POINT ( 'NONE',  ( 32.55216893130537414, -275.3040469787976576, -237.9255313598904706 ) ) ;
#77716=CARTESIAN_POINT ( 'NONE',  ( 26.06567488523061016, -275.9632682556931513, -314.1398373039746730 ) ) ;
#77717=CARTESIAN_POINT ( 'NONE',  ( -104.0479078780042954, -298.0317166746140174, -303.5168368878861997 ) ) ;
#77720=CARTESIAN_POINT ( 'NONE',  ( -106.0562381696035601, -294.2766238441584505, -302.2769093644306508 ) ) ;
#77721=CARTESIAN_POINT ( 'NONE',  ( 20.88216690037645407, -275.6795270999575678, -314.4969282740946142 ) ) ;
#77723=CARTESIAN_POINT ( 'NONE',  ( -69.23157864404510065, -287.3869056968936775, -203.5563443510324930 ) ) ;
#77724=CARTESIAN_POINT ( 'NONE',  ( 8.505167781035055441, -295.9570183292405545, -331.3592528217970425 ) ) ;
#77725=CARTESIAN_POINT ( 'NONE',  ( 29.12346494758562798, -294.2598354576129509, -232.2771246368934044 ) ) ;
#77726=CARTESIAN_POINT ( 'NONE',  ( -111.4346355418993113, -292.4160058650974747, -280.9535615949628777 ) ) ;
#77727=CARTESIAN_POINT ( 'NONE',  ( -112.1129699557743038, -276.5127736120763871, -273.4083514812512590 ) ) ;
#77729=CARTESIAN_POINT ( 'NONE',  ( -77.62120398176004699, -281.4274812970101038, -207.6987335635573686 ) ) ;
#77730=CARTESIAN_POINT ( 'NONE',  ( -110.3008771213403207, -294.4400511559276765, -285.1987532809184813 ) ) ;
#77731=CARTESIAN_POINT ( 'NONE',  ( -83.11775814082450609, -285.5313574879745033, -330.7996654721629852 ) ) ;
#77732=CARTESIAN_POINT ( 'NONE',  ( -46.75097764371336950, -284.8503500048736328, -197.6073663542804866 ) ) ;
#77733=CARTESIAN_POINT ( 'NONE',  ( -54.19524147295266658, -170.4633805983236243, -363.5514204490719976 ) ) ;
#77735=CARTESIAN_POINT ( 'NONE',  ( -106.1950888416815815, -283.8935605391519630, -294.8283413578931800 ) ) ;
#77736=ORIENTED_EDGE ( 'NONE', *, *, #13462, .F. ) ;
#77737=CARTESIAN_POINT ( 'NONE',  ( 0.7269116491058242868, -283.6365711119959201, -336.9516109343309722 ) ) ;
#77738=CARTESIAN_POINT ( 'NONE',  ( -99.01537480441263028, -283.9548576862641198, -224.8385612877828237 ) ) ;
#77740=CARTESIAN_POINT ( 'NONE',  ( -111.5068200340285358, -279.7427459786285908, -250.5023810691645565 ) ) ;
#77741=CARTESIAN_POINT ( 'NONE',  ( -12.07731067674798453, -278.2494985195435788, -342.4194524159306070 ) ) ;
#77742=CARTESIAN_POINT ( 'NONE',  ( -2.443822705920469573, -281.1529579519755657, -201.8230499438094228 ) ) ;
#77743=CARTESIAN_POINT ( 'NONE',  ( -21.33282851196157992, -271.7666405000204009, -200.3683826091710216 ) ) ;
#77744=CARTESIAN_POINT ( 'NONE',  ( -62.74176713377130454, -183.3418054874163374, -362.5124067139283852 ) ) ;
#77745=CARTESIAN_POINT ( 'NONE',  ( -63.98262090302324623, -275.7040825150743331, -200.4166767126971820 ) ) ;
#77746=CARTESIAN_POINT ( 'NONE',  ( 184.7839567310230393, 263.7331535000452050, -153.2007708629784304 ) ) ;
#77748=CARTESIAN_POINT ( 'NONE',  ( -57.53447368128914974, -277.8102896992081128, -198.4994543767004984 ) ) ;
#77749=CARTESIAN_POINT ( 'NONE',  ( 14.72725970433147502, -294.5331989152616643, -214.9463461217171130 ) ) ;
#77750=CARTESIAN_POINT ( 'NONE',  ( -39.70062654329873197, -294.4311075229616677, -343.4374290788379085 ) ) ;
#77751=CARTESIAN_POINT ( 'NONE',  ( -114.1260278879859413, -290.1207313203814806, -265.4934785606679384 ) ) ;
#77754=CARTESIAN_POINT ( 'NONE',  ( -61.42321264789228508, -293.9335327574731878, -342.9332408237028744 ) ) ;
#77755=CARTESIAN_POINT ( 'NONE',  ( -54.92743348445259244, -284.2222797707517543, -198.6341100497998582 ) ) ;
#77756=CARTESIAN_POINT ( 'NONE',  ( -73.24477305733812216, -293.4315744566847002, -205.3276969249216961 ) ) ;
#77758=CARTESIAN_POINT ( 'NONE',  ( -49.51719730274771791, -284.3741141461949837, -197.6285641248489071 ) ) ;
#77759=CARTESIAN_POINT ( 'NONE',  ( -104.5576213484313115, -285.4700433977267835, -300.0808658138208784 ) ) ;
#77760=CARTESIAN_POINT ( 'NONE',  ( -84.13244910653557440, -292.3681377695119750, -209.4381703824881242 ) ) ;
#77761=CARTESIAN_POINT ( 'NONE',  ( -64.07205397518960410, -283.9028455087408247, -338.3572695274557418 ) ) ;
#77762=CARTESIAN_POINT ( 'NONE',  ( -113.8382851596718268, -295.2850104998828442, -275.2984077688835214 ) ) ;
#77763=CIRCLE ( 'NONE', #56622, 1.895975569037589015 ) ;
#77764=CARTESIAN_POINT ( 'NONE',  ( -105.0089236347139945, -290.8833014963769870, -306.7658660648459090 ) ) ;
#77765=CARTESIAN_POINT ( 'NONE',  ( -73.13966934655017837, -290.0060818592173177, -338.4789626690590012 ) ) ;
#77766=CARTESIAN_POINT ( 'NONE',  ( 21.99033934664551282, -287.1233763233467471, -227.7469768085139208 ) ) ;
#77769=CARTESIAN_POINT ( 'NONE',  ( -110.3946422607836126, -298.1568118272001584, -290.4502475818501921 ) ) ;
#77770=CARTESIAN_POINT ( 'NONE',  ( -77.92658435468045752, -296.2037043965462999, -205.5061610055302310 ) ) ;
#77771=CARTESIAN_POINT ( 'NONE',  ( 23.88581452348766732, -280.0545185465205691, -230.0875585399231795 ) ) ;
#77772=CARTESIAN_POINT ( 'NONE',  ( 32.96099562826828588, -275.4590792988642534, -301.6190429368886612 ) ) ;
#77774=CARTESIAN_POINT ( 'NONE',  ( -105.3951433894272327, -295.4076314074646348, -242.0868078917496007 ) ) ;
#77775=CARTESIAN_POINT ( 'NONE',  ( 31.10348871756850286, -276.9383875020517962, -242.0623013506351811 ) ) ;
#77776=CARTESIAN_POINT ( 'NONE',  ( -37.12443831161420604, -296.2947748573664626, -196.3449554908045229 ) ) ;
#77777=CARTESIAN_POINT ( 'NONE',  ( -78.15788021377544226, -296.8192619657740465, -331.4238908116442417 ) ) ;
#77778=CARTESIAN_POINT ( 'NONE',  ( -10.36350882710902610, -295.7712887474172589, -338.5256488470991485 ) ) ;
#77780=CARTESIAN_POINT ( 'NONE',  ( -79.02216245182466992, -297.2043292419114096, -334.1512384923340164 ) ) ;
#77781=CARTESIAN_POINT ( 'NONE',  ( -74.84261421891243060, -295.5543429858998365, -205.1576297279182484 ) ) ;
#77782=CARTESIAN_POINT ( 'NONE',  ( -79.59637677992579086, -292.1159801070423327, -210.6464483809947694 ) ) ;
#77783=CARTESIAN_POINT ( 'NONE',  ( -70.07229665704188903, -274.4347458730334779, -200.8279102821391575 ) ) ;
#77784=CARTESIAN_POINT ( 'NONE',  ( -104.5935277712419378, -288.7264203095251673, -300.3628844216444804 ) ) ;
#77786=CARTESIAN_POINT ( 'NONE',  ( -44.04365173154280910, -274.4620505115028095, -193.6618427816122505 ) ) ;
#77787=CARTESIAN_POINT ( 'NONE',  ( -106.0056192413246805, -296.5527686162330383, -295.3563757769372842 ) ) ;
#77788=CARTESIAN_POINT ( 'NONE',  ( 14.02138225634661417, -282.7481880881042571, -215.1514332593396546 ) ) ;
#77789=CARTESIAN_POINT ( 'NONE',  ( 36.13084604322573767, -279.9672099008169539, -248.9814357734026942 ) ) ;
#77790=CARTESIAN_POINT ( 'NONE',  ( -9.256782621126726340, -276.0430502786781517, -341.9470816572583090 ) ) ;
#77791=CARTESIAN_POINT ( 'NONE',  ( 37.87485366581713464, -280.1072722916130147, -282.6453787612191491 ) ) ;
#77792=CARTESIAN_POINT ( 'NONE',  ( 27.71294056767867175, -279.0503911189208566, -232.7058109421343488 ) ) ;
#77793=CARTESIAN_POINT ( 'NONE',  ( 0.9343157785141926741, -273.1485294302837588, -207.5095346831271002 ) ) ;
#77794=CARTESIAN_POINT ( 'NONE',  ( -96.36765988166499142, -281.1874927779224436, -224.0705127729911226 ) ) ;
#77796=CARTESIAN_POINT ( 'NONE',  ( 145.2857639756989272, -297.1570670221753971, -195.3611179825600175 ) ) ;
#77797=CARTESIAN_POINT ( 'NONE',  ( -33.37747646669512847, -296.3410002000283612, -194.3756134808325555 ) ) ;
#77798=CARTESIAN_POINT ( 'NONE',  ( -40.53689108001209718, -290.0322976746473387, -195.0607842498029356 ) ) ;
#77799=CARTESIAN_POINT ( 'NONE',  ( -44.89704630020091969, -291.9591444340095450, -193.6797626336525298 ) ) ;
#77800=CARTESIAN_POINT ( 'NONE',  ( -15.10710243309569023, -278.7651667265386664, -342.2184831078598677 ) ) ;
#77801=CARTESIAN_POINT ( 'NONE',  ( 30.91656252957844586, -273.1427144208873870, -239.1579048482124961 ) ) ;
#77803=CARTESIAN_POINT ( 'NONE',  ( -4.762154311256177941, -284.5465915205719512, -338.5507551766988286 ) ) ;
#77805=CARTESIAN_POINT ( 'NONE',  ( -6.484393732722012693, -284.4572015869234747, -201.9891716034530020 ) ) ;
#77807=CARTESIAN_POINT ( 'NONE',  ( -28.86527586023586167, -293.7373616666228600, -343.3183801584384582 ) ) ;
#77808=CARTESIAN_POINT ( 'NONE',  ( 34.91802828742577702, -285.4703453651744667, -253.2944313378754373 ) ) ;
#77810=CARTESIAN_POINT ( 'NONE',  ( -12.36558361046928489, -292.7272644521042935, -341.1349493831488076 ) ) ;
#77811=CARTESIAN_POINT ( 'NONE',  ( -80.52970607768872924, -283.9585459959500326, -207.3886543045527162 ) ) ;
#77812=CARTESIAN_POINT ( 'NONE',  ( -62.60171197721145830, -281.3181546951419705, -200.9647420576450543 ) ) ;
#77813=CARTESIAN_POINT ( 'NONE',  ( -26.69157130273216438, -287.3896862812131303, -194.4489248195647804 ) ) ;
#77814=CARTESIAN_POINT ( 'NONE',  ( 27.42935362671035904, -280.3192388539116564, -310.1934510155680869 ) ) ;
#77815=CARTESIAN_POINT ( 'NONE',  ( 6.926924441421244971, -286.6736382773327136, -212.2516743373252837 ) ) ;
#77816=CARTESIAN_POINT ( 'NONE',  ( -70.01814581552230266, -281.0382979637683434, -204.4106375890868037 ) ) ;
#77817=CARTESIAN_POINT ( 'NONE',  ( 13.43984192653332066, -281.5876297188358421, -217.6233023206523853 ) ) ;
#77818=CARTESIAN_POINT ( 'NONE',  ( -69.12262362710320929, -287.6161643423073997, -202.0215156371622811 ) ) ;
#77820=CARTESIAN_POINT ( 'NONE',  ( -114.3417001280813849, -272.5521521680024648, -270.3611179825603017 ) ) ;
#77821=CARTESIAN_POINT ( 'NONE',  ( -71.91262985746872971, -291.4913419672820396, -336.5321709462367608 ) ) ;
#77823=CARTESIAN_POINT ( 'NONE',  ( 13.84574458161073096, -290.9090924074130839, -334.4957818155094174 ) ) ;
#77825=CARTESIAN_POINT ( 'NONE',  ( 1.493147996876710737, -272.5697584191618148, -206.0036553438961846 ) ) ;
#77826=CARTESIAN_POINT ( 'NONE',  ( -96.79618238036371736, -294.3065505336375054, -318.0431316831548543 ) ) ;
#77827=CARTESIAN_POINT ( 'NONE',  ( -105.5082903411829562, -272.2547354049543173, -243.8168174096828977 ) ) ;
#77828=CARTESIAN_POINT ( 'NONE',  ( 10.58068572582067901, -289.8964943967174008, -326.4121095182097179 ) ) ;
#77830=CARTESIAN_POINT ( 'NONE',  ( 32.93175798253300712, -283.0062388817232204, -246.9701215346832441 ) ) ;
#77832=CARTESIAN_POINT ( 'NONE',  ( -95.92750843724100207, -291.3119246698091729, -319.4355536755416551 ) ) ;
#77833=CARTESIAN_POINT ( 'NONE',  ( -95.07508638284664926, -291.1843557862740113, -320.5622572649332369 ) ) ;
#77834=CARTESIAN_POINT ( 'NONE',  ( -42.84564067182729730, -287.9828744997710714, -195.5503704792633357 ) ) ;
#77835=CARTESIAN_POINT ( 'NONE',  ( -93.07521974658013164, -279.4458976767204490, -217.1551422781808469 ) ) ;
#77836=CARTESIAN_POINT ( 'NONE',  ( 5.771916914311491453, -292.5531352304536767, -332.4774978167889685 ) ) ;
#77837=CARTESIAN_POINT ( 'NONE',  ( 37.19127262340634843, -281.6274672583128336, -289.6959564187018259 ) ) ;
#77838=CARTESIAN_POINT ( 'NONE',  ( -6.029159428263385578, -276.3285712387122430, -203.0529440475563092 ) ) ;
#77839=CARTESIAN_POINT ( 'NONE',  ( -37.37352853689063181, -276.5519495502701375, -200.3611179825600459 ) ) ;
#77840=CARTESIAN_POINT ( 'NONE',  ( -1.959709683981272210, -274.8299380774016640, -337.6075957189154906 ) ) ;
#77842=CARTESIAN_POINT ( 'NONE',  ( 35.74908926908865681, -281.0364354699721616, -268.5883340753606490 ) ) ;
#77843=CARTESIAN_POINT ( 'NONE',  ( -99.31941938901326239, -279.1565484298548085, -315.4030906218728774 ) ) ;
#77844=CARTESIAN_POINT ( 'NONE',  ( -67.27358702228808340, -274.9664237572079628, -203.2256083818994057 ) ) ;
#77845=CARTESIAN_POINT ( 'NONE',  ( -113.2529073734491902, -283.7584975083096310, -258.5956698820859856 ) ) ;
#77846=CARTESIAN_POINT ( 'NONE',  ( -77.82794896661859241, -293.2602204306523390, -208.4027636859447910 ) ) ;
#77847=CARTESIAN_POINT ( 'NONE',  ( -98.93259805941819707, -274.7549802943333361, -225.4071067310807166 ) ) ;
#77848=CARTESIAN_POINT ( 'NONE',  ( -102.3091655580507506, -274.3992959762760506, -229.9565797758355359 ) ) ;
#77850=CARTESIAN_POINT ( 'NONE',  ( -13.78740676530620846, -276.5712360821904099, -339.5098068145924231 ) ) ;
#77851=CARTESIAN_POINT ( 'NONE',  ( -109.6127013934152927, -298.8030332293877791, -250.8969695909260622 ) ) ;
#77852=CARTESIAN_POINT ( 'NONE',  ( -94.64290160504012306, -283.2188028014856513, -222.2300392587783335 ) ) ;
#77853=CARTESIAN_POINT ( 'NONE',  ( -7.194570306159838502, -292.1036285232881937, -199.5167577954833860 ) ) ;
#77854=CARTESIAN_POINT ( 'NONE',  ( 34.47356654315331781, -273.8360046415699003, -290.7650038886256425 ) ) ;
#77855=CARTESIAN_POINT ( 'NONE',  ( -36.07944315171685901, -290.6367294326320234, -346.5636392002280104 ) ) ;
#77856=CARTESIAN_POINT ( 'NONE',  ( -107.2924645115570712, -289.7624593109689499, -248.3844847533809173 ) ) ;
#77858=CARTESIAN_POINT ( 'NONE',  ( 27.56153710021769498, -291.5941862183674402, -229.9352296556147621 ) ) ;
#77859=CARTESIAN_POINT ( 'NONE',  ( -108.6842922323005638, -290.0128686932682172, -285.9859576085128197 ) ) ;
#77861=CARTESIAN_POINT ( 'NONE',  ( 28.64480375442017035, -289.1430128325756073, -309.4414687295179647 ) ) ;
#77862=CARTESIAN_POINT ( 'NONE',  ( -110.3724700157753205, -278.9177369472043324, -267.9117865372344909 ) ) ;
#77863=CARTESIAN_POINT ( 'NONE',  ( -68.11481489992183924, -294.3672165408218575, -340.6071706671751258 ) ) ;
#77864=CARTESIAN_POINT ( 'NONE',  ( -83.81499226946739611, -284.3225493125258936, -331.6941910696224340 ) ) ;
#77865=CARTESIAN_POINT ( 'NONE',  ( -114.1869479316844291, -284.8183872267521792, -275.7205382013739836 ) ) ;
#77866=CARTESIAN_POINT ( 'NONE',  ( -40.23094732082699920, -283.4227500178218406, -343.3250798918173814 ) ) ;
#77867=CARTESIAN_POINT ( 'NONE',  ( 45.21095933465400662, 12.48609948641568401, -332.0833974251048630 ) ) ;
#77869=CARTESIAN_POINT ( 'NONE',  ( -32.31571139608886511, -123.7737035626091142, -363.2393823568430662 ) ) ;
#77870=CARTESIAN_POINT ( 'NONE',  ( 102.0852645817304420, 115.1042933526224346, -279.6109006776878232 ) ) ;
#77871=CARTESIAN_POINT ( 'NONE',  ( 33.05043141068819068, -275.0128741221709561, -290.3455852157211439 ) ) ;
#77872=CARTESIAN_POINT ( 'NONE',  ( -3.951671187673817975, -273.4236201873168284, -205.0834662887545505 ) ) ;
#77873=CARTESIAN_POINT ( 'NONE',  ( 4.188801008173478557, -294.0164634293062136, -335.1906872579032779 ) ) ;
#77874=CARTESIAN_POINT ( 'NONE',  ( 154.3500357470443021, 204.3678965669933802, -214.6393225715670781 ) ) ;
#77876=CARTESIAN_POINT ( 'NONE',  ( 36.75691449646658526, -274.4768550205615156, -289.4056338577922247 ) ) ;
#77877=CARTESIAN_POINT ( 'NONE',  ( -37.85442852042710626, -299.9060784993138782, -196.1276848580625938 ) ) ;
#77879=CARTESIAN_POINT ( 'NONE',  ( -90.04807432586440541, -292.3649870685533187, -219.4075686216673660 ) ) ;
#77881=CARTESIAN_POINT ( 'NONE',  ( -93.49883429147621428, -298.2097262211927386, -217.9462348266160632 ) ) ;
#77883=CARTESIAN_POINT ( 'NONE',  ( 34.62691000563234667, -287.8747988460855822, -257.4858968189267330 ) ) ;
#77884=CARTESIAN_POINT ( 'NONE',  ( -110.1893635948897838, -297.0465562167128155, -294.8024098420250994 ) ) ;
#77885=CARTESIAN_POINT ( 'NONE',  ( -27.74928510507582757, -295.4259222851308664, -346.7525137249320437 ) ) ;
#77886=CARTESIAN_POINT ( 'NONE',  ( 30.82763263933218312, -293.3700666634761092, -244.2470973320261862 ) ) ;
#77890=CARTESIAN_POINT ( 'NONE',  ( 19.74860421915299824, -278.1540587828893649, -319.8782978123292651 ) ) ;
#77892=CARTESIAN_POINT ( 'NONE',  ( -28.22606646958156773, -279.6724005652288270, -193.9109903708342131 ) ) ;
#77893=CARTESIAN_POINT ( 'NONE',  ( 32.28177383408095125, -276.1910163916273859, -247.4828649506638669 ) ) ;
#77894=CARTESIAN_POINT ( 'NONE',  ( 29.05108971108531435, -276.8255565761799062, -233.2939253991620205 ) ) ;
#77895=CARTESIAN_POINT ( 'NONE',  ( -35.77161143971162716, -275.0526921226901322, -345.7128069339277658 ) ) ;
#77896=CARTESIAN_POINT ( 'NONE',  ( -55.32675472505136582, -298.4661548596025114, -199.4537364939857582 ) ) ;
#77897=CARTESIAN_POINT ( 'NONE',  ( -70.00176890781557404, -294.0658395143611301, -336.3057525351154027 ) ) ;
#77899=CARTESIAN_POINT ( 'NONE',  ( -86.76999003683769729, -279.8786128753487787, -211.3309135519273241 ) ) ;
#77900=CARTESIAN_POINT ( 'NONE',  ( 20.83820548198987765, -276.3384477307179168, -314.4530513460756538 ) ) ;
#77902=CARTESIAN_POINT ( 'NONE',  ( -15.53786412000536998, -285.0132759303832586, -196.9719709206454752 ) ) ;
#77903=CARTESIAN_POINT ( 'NONE',  ( -33.47854310738762962, -300.1005598813350161, -195.1931292090783359 ) ) ;
#77905=CARTESIAN_POINT ( 'NONE',  ( 35.28327639339224930, -286.8657237183146549, -279.2050148687105207 ) ) ;
#77908=CARTESIAN_POINT ( 'NONE',  ( -86.13564841907148661, -277.6042543601321881, -214.7093020070257126 ) ) ;
#77909=CARTESIAN_POINT ( 'NONE',  ( -103.8950534298601553, -277.5491990153288953, -238.8403564528508127 ) ) ;
#77910=CARTESIAN_POINT ( 'NONE',  ( -107.5396999278674173, -282.3069433636513281, -295.2848038767965022 ) ) ;
#77911=CARTESIAN_POINT ( 'NONE',  ( -33.28594586776748088, -288.1032519430545449, -195.4204966776122205 ) ) ;
#77912=CARTESIAN_POINT ( 'NONE',  ( -85.35345359285548739, -278.9378994995622065, -325.9442114815389004 ) ) ;
#77914=CARTESIAN_POINT ( 'NONE',  ( -95.05656618886520448, -293.2136646671236235, -222.4455957921904314 ) ) ;
#77915=CARTESIAN_POINT ( 'NONE',  ( -25.94437624670307230, -275.1487687691954420, -345.4881771570215960 ) ) ;
#77916=CARTESIAN_POINT ( 'NONE',  ( -40.50188109374197154, -277.7443176950906718, -343.4071943015082411 ) ) ;
#77917=CARTESIAN_POINT ( 'NONE',  ( 36.44992186715253268, -283.3689571388582067, -256.0494111413789255 ) ) ;
#77919=CARTESIAN_POINT ( 'NONE',  ( -4.928195225406174274, -290.5488790721537384, -338.6298449423319994 ) ) ;
#77920=CARTESIAN_POINT ( 'NONE',  ( -94.33683259953144784, -295.2274073608895719, -221.5918554959565938 ) ) ;
#77922=CARTESIAN_POINT ( 'NONE',  ( 19.39014416156286558, -273.5793335152262671, -223.6413007421882924 ) ) ;
#77923=CARTESIAN_POINT ( 'NONE',  ( -19.75697806506245158, -290.4200668121802664, -198.1855433051566422 ) ) ;
#77926=CARTESIAN_POINT ( 'NONE',  ( -95.12312225120990661, -289.7113846199916338, -220.5012585941549901 ) ) ;
#77927=CARTESIAN_POINT ( 'NONE',  ( 37.56182725202084072, -285.6290270329834016, -257.5002479405208646 ) ) ;
#77928=CARTESIAN_POINT ( 'NONE',  ( -54.91449638041446946, -287.2471936631757785, -198.8481140307592341 ) ) ;
#77929=CARTESIAN_POINT ( 'NONE',  ( -65.16407879324741259, -286.4820148051673527, -202.6424477915757052 ) ) ;
#77930=CARTESIAN_POINT ( 'NONE',  ( -41.97849182923987854, -293.9738672472051917, -195.1487056649911551 ) ) ;
#77931=CARTESIAN_POINT ( 'NONE',  ( 36.23835796270876131, -273.4123459145749848, -253.1207721556502577 ) ) ;
#77932=CARTESIAN_POINT ( 'NONE',  ( 29.92699025259534906, -275.3989262285777500, -232.8260239804113496 ) ) ;
#77933=CARTESIAN_POINT ( 'NONE',  ( -112.9494946530976023, -288.6214560481333251, -271.1881267596637031 ) ) ;
#77934=CARTESIAN_POINT ( 'NONE',  ( -20.12610442838468217, -276.8369733285863390, -345.4666413788748969 ) ) ;
#77935=CARTESIAN_POINT ( 'NONE',  ( -107.5252555960994840, -298.1991143452128767, -295.9317583000727154 ) ) ;
#77937=CARTESIAN_POINT ( 'NONE',  ( -108.5753225508914852, -282.9998984035043463, -288.4446606620529110 ) ) ;
#77938=CARTESIAN_POINT ( 'NONE',  ( -61.38180560496080318, -277.7399057772449851, -199.2635913898405704 ) ) ;
#77940=CARTESIAN_POINT ( 'NONE',  ( -32.70521247465042336, -272.5894392137715272, -194.1824063602071533 ) ) ;
#77941=CARTESIAN_POINT ( 'NONE',  ( -51.30847225048231053, -276.5840573300928895, -342.1164100823701801 ) ) ;
#77942=CARTESIAN_POINT ( 'NONE',  ( -5.221979995643446060, -296.1416882902084353, -336.7002557253854889 ) ) ;
#77943=CARTESIAN_POINT ( 'NONE',  ( -8.962664155152358703, -279.3351107549164567, -199.1142034729891179 ) ) ;
#77944=CARTESIAN_POINT ( 'NONE',  ( -95.78488004436138681, -296.8751655969617218, -314.5156954167891854 ) ) ;
#77945=CARTESIAN_POINT ( 'NONE',  ( -86.06827166205630419, -297.0268035059925751, -329.3443316791561983 ) ) ;
#77946=CARTESIAN_POINT ( 'NONE',  ( -37.14748037964942284, -297.8879779239914569, -197.3582748454228408 ) ) ;
#77947=CARTESIAN_POINT ( 'NONE',  ( -101.4335920447371109, -293.0744354842524331, -231.4094808189903176 ) ) ;
#77949=CARTESIAN_POINT ( 'NONE',  ( -69.79477315177382479, -285.8032460596815554, -200.5198374910926020 ) ) ;
#77950=CARTESIAN_POINT ( 'NONE',  ( 7.490776091255906266, -274.5878949043317334, -331.5026876122603881 ) ) ;
#77951=CARTESIAN_POINT ( 'NONE',  ( 37.14387511131583608, -287.6297729102961398, -289.8777541112779659 ) ) ;
#77952=CARTESIAN_POINT ( 'NONE',  ( -90.66585033668808080, -281.2720822623585377, -218.0539240777975181 ) ) ;
#77953=CARTESIAN_POINT ( 'NONE',  ( -27.79404683961005418, -285.2351210192896929, -197.7508517356553739 ) ) ;
#77954=CARTESIAN_POINT ( 'NONE',  ( -98.26104027413573760, -287.9564642711482634, -314.1305269378204343 ) ) ;
#77955=CARTESIAN_POINT ( 'NONE',  ( -89.67076919512652466, -242.4121354169174367, -340.4712336312485377 ) ) ;
#77956=CARTESIAN_POINT ( 'NONE',  ( 33.44974758320255859, -286.8208786887635711, -252.2396500136737245 ) ) ;
#77958=CARTESIAN_POINT ( 'NONE',  ( -33.05985201258903317, -283.9407356820760242, -347.0194082359944332 ) ) ;
#77959=CARTESIAN_POINT ( 'NONE',  ( -96.88010299293385685, -289.1794479861563900, -224.4577660744706691 ) ) ;
#77960=CARTESIAN_POINT ( 'NONE',  ( -44.86202929437367715, -291.0180442021259637, -193.9129069774049299 ) ) ;
#77961=CARTESIAN_POINT ( 'NONE',  ( -109.7954413275817416, -280.4541711175155001, -246.5948669354799563 ) ) ;
#77962=CARTESIAN_POINT ( 'NONE',  ( -97.32078551127240473, -280.5069482343954519, -222.8657751399411779 ) ) ;
#77963=CARTESIAN_POINT ( 'NONE',  ( 9.278169557086753727, -280.5465787402499700, -214.1206034837695711 ) ) ;
#77964=CARTESIAN_POINT ( 'NONE',  ( 32.98510210217236249, -277.2140611195449651, -244.3007738723994180 ) ) ;
#77965=CARTESIAN_POINT ( 'NONE',  ( -77.08222869163832058, -295.5688350394901818, -336.3753312726047966 ) ) ;
#77966=CARTESIAN_POINT ( 'NONE',  ( -106.6494327325996778, -288.2078448062795246, -298.2179161902017768 ) ) ;
#77968=CARTESIAN_POINT ( 'NONE',  ( -80.34717540523259061, -294.5707566997787126, -329.7307665325215567 ) ) ;
#77971=CARTESIAN_POINT ( 'NONE',  ( -65.84489675661505714, -285.3480853791600111, -339.1418494308663298 ) ) ;
#77972=CARTESIAN_POINT ( 'NONE',  ( -110.2630065774707049, -296.1685290390551586, -274.1782572788544030 ) ) ;
#77973=CARTESIAN_POINT ( 'NONE',  ( -42.04878047327095913, -293.0737918267600435, -193.8148188907349549 ) ) ;
#77974=CARTESIAN_POINT ( 'NONE',  ( -45.64281653973429087, -283.8114164703379743, -343.0412688852480301 ) ) ;
#77976=CARTESIAN_POINT ( 'NONE',  ( 31.04612929369649166, -274.1604457384432294, -235.4910018475604829 ) ) ;
#77977=CARTESIAN_POINT ( 'NONE',  ( -44.89530065077337184, -292.6104526181504184, -193.7820876729325619 ) ) ;
#77978=CARTESIAN_POINT ( 'NONE',  ( -92.99603803810333602, -283.4038404328582033, -218.8751118250499985 ) ) ;
#77979=CARTESIAN_POINT ( 'NONE',  ( -92.79979941882028527, -291.6171577397007582, -216.8985433687288946 ) ) ;
#77980=CARTESIAN_POINT ( 'NONE',  ( 35.65132491270625792, -287.9302143546821640, -273.7565812421768214 ) ) ;
#77983=CARTESIAN_POINT ( 'NONE',  ( 45.23250845692812305, 11.08492981906800701, -328.3308289300945830 ) ) ;
#77984=CARTESIAN_POINT ( 'NONE',  ( 17.34304175893838007, -283.8092021542565817, -323.6558720886995957 ) ) ;
#77985=CARTESIAN_POINT ( 'NONE',  ( 10.64812456238590777, -284.1952119285918457, -210.2361428286349110 ) ) ;
#77987=CARTESIAN_POINT ( 'NONE',  ( -34.28674091711881289, -279.0117505499570711, -197.1030895341135931 ) ) ;
#77988=CARTESIAN_POINT ( 'NONE',  ( 27.62870382355426102, -275.7612537966296600, -311.7468852477241512 ) ) ;
#77989=CARTESIAN_POINT ( 'NONE',  ( -111.0885591932006520, -280.3878400200118222, -283.1421908959335383 ) ) ;
#77990=CARTESIAN_POINT ( 'NONE',  ( 155.0569925984352437, 204.5026487299929272, -215.2223648592982101 ) ) ;
#77992=CARTESIAN_POINT ( 'NONE',  ( 5.866126571937878786, -279.2002729723147354, -207.3397723647147188 ) ) ;
#77993=CARTESIAN_POINT ( 'NONE',  ( -96.23967892941550417, -283.2044057919530360, -224.4832575617479051 ) ) ;
#77994=CARTESIAN_POINT ( 'NONE',  ( -112.9328559201644566, -298.2141660918381945, -278.1039326154722175 ) ) ;
#77995=CARTESIAN_POINT ( 'NONE',  ( 28.79155699555532166, -293.6239379426692153, -239.1872575319255532 ) ) ;
#77997=CARTESIAN_POINT ( 'NONE',  ( -110.6157490441761411, -289.1544942125172497, -276.6555871042371564 ) ) ;
#77998=CARTESIAN_POINT ( 'NONE',  ( 31.15573365154443408, -275.7528545977390309, -235.4123790656805681 ) ) ;
#77999=CARTESIAN_POINT ( 'NONE',  ( -69.49096092639894096, -273.6167721611693082, -204.8216258413955302 ) ) ;
#78004=CARTESIAN_POINT ( 'NONE',  ( 35.73836176923398966, -282.7159446937331495, -276.7645155475801744 ) ) ;
#78005=CARTESIAN_POINT ( 'NONE',  ( 0.8450743835883158805, -282.3139502053393812, -204.6068958529008057 ) ) ;
#78006=CARTESIAN_POINT ( 'NONE',  ( -66.66475680542281168, -282.5046936961529696, -337.4833533606856122 ) ) ;
#78007=CARTESIAN_POINT ( 'NONE',  ( 16.13297601197039555, -282.6807190127457261, -218.7966961930482057 ) ) ;
#78008=CARTESIAN_POINT ( 'NONE',  ( 5.787031647423192204, -274.9358990430971517, -330.1787889949113719 ) ) ;
#78009=CYLINDRICAL_SURFACE ( 'NONE', #85087, 2.395975569037589459 ) ;
#78011=CARTESIAN_POINT ( 'NONE',  ( -38.53218329042907442, -277.8695521315996189, -347.1904194959677739 ) ) ;
#78015=CARTESIAN_POINT ( 'NONE',  ( -98.43975039623825296, -285.9334007008319531, -314.5553682605402628 ) ) ;
#78016=CARTESIAN_POINT ( 'NONE',  ( 31.68901697243846272, -293.0728598703734633, -294.7482962532113788 ) ) ;
#78017=CARTESIAN_POINT ( 'NONE',  ( 37.40337367037867722, -287.1276814807554842, -288.4856632237528515 ) ) ;
#78018=CARTESIAN_POINT ( 'NONE',  ( -82.07344192543625638, -283.6724660893178225, -211.3946420260229786 ) ) ;
#78019=CARTESIAN_POINT ( 'NONE',  ( -110.6844972590510565, -283.0481292776624400, -276.3785115289605301 ) ) ;
#78020=CARTESIAN_POINT ( 'NONE',  ( -61.60811762394020974, -287.6116653174140083, -340.2833247160724568 ) ) ;
#78021=CARTESIAN_POINT ( 'NONE',  ( -36.17189450360240954, -284.2422398756755797, -343.7488694187027818 ) ) ;
#78022=CARTESIAN_POINT ( 'NONE',  ( 8.313569684162438023, -272.6768079095342614, -210.8582022216696430 ) ) ;
#78023=CARTESIAN_POINT ( 'NONE',  ( -43.58023711589384419, -284.3745917571832251, -194.3642154339628405 ) ) ;
#78024=CARTESIAN_POINT ( 'NONE',  ( -51.45003256453077967, -299.8720352404391178, -196.6471005666851397 ) ) ;
#78025=CARTESIAN_POINT ( 'NONE',  ( -108.2393916541987267, -282.8746962262992497, -245.3902196875901325 ) ) ;
#78026=CARTESIAN_POINT ( 'NONE',  ( -24.84799789795610891, -281.1567151623135032, -198.1993839950561380 ) ) ;
#78027=CARTESIAN_POINT ( 'NONE',  ( 28.76282144291930010, -290.0276912174375070, -306.2502114654001844 ) ) ;
#78030=CARTESIAN_POINT ( 'NONE',  ( 5.812028816583048041, -296.3928250819216714, -332.4496372304887473 ) ) ;
#78032=CARTESIAN_POINT ( 'NONE',  ( -104.9445066263934336, -276.1229172585535139, -302.9599979713765947 ) ) ;
#78033=CARTESIAN_POINT ( 'NONE',  ( -88.53427863837782752, -290.5526114677807072, -213.0594711866723969 ) ) ;
#78034=CARTESIAN_POINT ( 'NONE',  ( -47.92771635643258321, -293.5887522324441079, -343.4497788984960494 ) ) ;
#78035=CARTESIAN_POINT ( 'NONE',  ( -71.15374545444680621, -278.2809459688517109, -205.0936680473996603 ) ) ;
#78036=CARTESIAN_POINT ( 'NONE',  ( -111.6239364621605574, -270.7041710373114825, -264.7816375358765981 ) ) ;
#78037=CARTESIAN_POINT ( 'NONE',  ( 34.55348230529268960, -295.0678418764408093, -285.6637969265142942 ) ) ;
#78038=CARTESIAN_POINT ( 'NONE',  ( -54.49178911615188525, -288.3376638359845288, -195.3683826091709363 ) ) ;
#78039=CARTESIAN_POINT ( 'NONE',  ( -89.12347088402501072, -295.8198303883943936, -214.2417575089994841 ) ) ;
#78040=CARTESIAN_POINT ( 'NONE',  ( 18.44349158545691125, -289.8340234761826082, -318.7538335018079465 ) ) ;
#78041=CARTESIAN_POINT ( 'NONE',  ( -37.76657183856354294, -290.2867648098452378, -194.3756358058248566 ) ) ;
#78042=CARTESIAN_POINT ( 'NONE',  ( -96.22900833525611120, -291.3626350569492729, -314.5144402165781798 ) ) ;
#78044=CARTESIAN_POINT ( 'NONE',  ( -55.06133827327901287, -292.6212219061191036, -199.3779076407261641 ) ) ;
#78045=DIRECTION ( 'NONE',  ( 1.000000000000000000, 0.000000000000000000, 0.000000000000000000 ) ) ;
#78046=CARTESIAN_POINT ( 'NONE',  ( -101.3606066848042104, -292.3141433312226809, -228.1994284328014544 ) ) ;
#78047=CARTESIAN_POINT ( 'NONE',  ( 32.04141589397940493, -279.9561610777213332, -299.8947781878780461 ) ) ;
#78048=CARTESIAN_POINT ( 'NONE',  ( -3.636257387683622166, -292.5100513929653516, -205.6081788239876857 ) ) ;
#78049=CARTESIAN_POINT ( 'NONE',  ( 38.87126650710599307, -281.6894854985901588, -281.3421797100900221 ) ) ;
#78050=CARTESIAN_POINT ( 'NONE',  ( 29.27041051114071024, -280.7170019708249242, -231.7791143067110511 ) ) ;
#78051=CARTESIAN_POINT ( 'NONE',  ( -61.87961827879398413, -287.3716847475225791, -341.0570796647887732 ) ) ;
#78052=CARTESIAN_POINT ( 'NONE',  ( 22.33584591161826438, -279.0827678749289475, -226.1870705725358448 ) ) ;
#78053=CARTESIAN_POINT ( 'NONE',  ( -104.8670900613770982, -282.9819557755931214, -237.7218416429464014 ) ) ;
#78054=CARTESIAN_POINT ( 'NONE',  ( 21.44901790306999700, -279.3722026598804860, -221.7158794859921045 ) ) ;
#78055=CARTESIAN_POINT ( 'NONE',  ( 26.88642267267063346, -285.9197277107601280, -228.4535917965323506 ) ) ;
#78057=CARTESIAN_POINT ( 'NONE',  ( 13.43902604296970260, -294.3775230667600340, -216.8096636284770682 ) ) ;
#78058=CARTESIAN_POINT ( 'NONE',  ( 26.42873537441102982, -276.4195853971948509, -228.2667258571102309 ) ) ;
#78059=CARTESIAN_POINT ( 'NONE',  ( -94.47223206747702307, -277.5766073369651394, -315.8584469437942630 ) ) ;
#78060=CARTESIAN_POINT ( 'NONE',  ( -101.6851289270089183, -291.2759151002916269, -227.9697699020849768 ) ) ;
#78061=CARTESIAN_POINT ( 'NONE',  ( -52.65022701274669004, -281.3264997077161524, -344.4075889059903943 ) ) ;
#78062=CARTESIAN_POINT ( 'NONE',  ( -110.6028678928897335, -289.6361073270563224, -268.4436776839389722 ) ) ;
#78063=CARTESIAN_POINT ( 'NONE',  ( -44.62737072644875980, -293.1440563135716388, -345.0584305643869811 ) ) ;
#78066=CARTESIAN_POINT ( 'NONE',  ( 16.78798984941439443, -292.3565922022360155, -221.2158878559043842 ) ) ;
#78068=CARTESIAN_POINT ( 'NONE',  ( -92.05005921254146983, -270.6952119285918457, -226.6919474004047572 ) ) ;
#78069=CARTESIAN_POINT ( 'NONE',  ( -93.48246105589508659, -296.3275259632841880, -217.9286993795860212 ) ) ;
#78070=CARTESIAN_POINT ( 'NONE',  ( 34.16983101757539032, -279.3691288536743969, -245.1761672046240790 ) ) ;
#78071=CARTESIAN_POINT ( 'NONE',  ( -102.4893226013559371, -285.3396367682113919, -310.4745266897137981 ) ) ;
#78072=CARTESIAN_POINT ( 'NONE',  ( 19.51652875285404676, -286.7379501504116774, -224.5576706834501977 ) ) ;
#78073=CARTESIAN_POINT ( 'NONE',  ( -16.16327066967548021, -278.2935859473080882, -340.9992073342293111 ) ) ;
#78074=CARTESIAN_POINT ( 'NONE',  ( -64.18348173831088843, -293.4240369830604891, -340.0676365198945064 ) ) ;
#78075=CARTESIAN_POINT ( 'NONE',  ( -47.91595552745854292, -296.9484807267889437, -343.6671803159232468 ) ) ;
#78076=CARTESIAN_POINT ( 'NONE',  ( 5.616831537261391283, -275.2508945685091817, -329.9360129651079205 ) ) ;
#78079=CARTESIAN_POINT ( 'NONE',  ( -106.4924653643163452, -296.6533104477818483, -236.5392913216862212 ) ) ;
#78080=CARTESIAN_POINT ( 'NONE',  ( 21.51069490846390408, -290.1020244241570936, -315.9636680769573900 ) ) ;
#78081=CARTESIAN_POINT ( 'NONE',  ( 202.0873885898396338, 295.7612547068911226, -54.00000000005271517 ) ) ;
#78082=CARTESIAN_POINT ( 'NONE',  ( 22.04934442253710003, -288.7985424882168104, -312.9826676442696680 ) ) ;
#78083=EDGE_CURVE ( 'NONE', #65957, #47026, #59077, .T. ) ;
#78085=CARTESIAN_POINT ( 'NONE',  ( -64.64738932163504614, -278.7630909172327165, -198.5609388446419814 ) ) ;
#78086=CARTESIAN_POINT ( 'NONE',  ( -86.32400088434911822, -296.3631495316701034, -329.6405157434542730 ) ) ;
#78087=CARTESIAN_POINT ( 'NONE',  ( -112.4385296479938035, -288.8242006916239575, -259.9394053488470604 ) ) ;
#78088=CARTESIAN_POINT ( 'NONE',  ( -77.06767906920180167, -295.9020624739444543, -336.3593935745793146 ) ) ;
#78089=CARTESIAN_POINT ( 'NONE',  ( 27.17874114803742458, -294.3523879368091229, -304.6627473358265092 ) ) ;
#78093=CARTESIAN_POINT ( 'NONE',  ( 33.40684426212698099, -289.4401213434811098, -299.0913033591211274 ) ) ;
#78094=CARTESIAN_POINT ( 'NONE',  ( 44.71564893372296723, -278.0519495502701375, -270.3284710469131937 ) ) ;
#78096=CARTESIAN_POINT ( 'NONE',  ( 8.492444172443342154, -280.0097280366674113, -208.5491200923931672 ) ) ;
#78097=CARTESIAN_POINT ( 'NONE',  ( 6.690891535007532198, -284.4519230596821444, -330.8686323516036509 ) ) ;
#78098=CARTESIAN_POINT ( 'NONE',  ( 15.90171716690819892, -285.3637075533840743, -215.5546876419895455 ) ) ;
#78099=CARTESIAN_POINT ( 'NONE',  ( -91.65993919530676237, -287.9130770110612048, -321.3367461437783277 ) ) ;
#78100=CARTESIAN_POINT ( 'NONE',  ( 16.10102229784061834, -278.1648091990335274, -324.1389714895616407 ) ) ;
#78102=CARTESIAN_POINT ( 'NONE',  ( -96.40570294426359510, -279.1525450687675516, -227.4607267101017385 ) ) ;
#78103=CARTESIAN_POINT ( 'NONE',  ( -34.30079519696562329, -279.4399395265006660, -197.3098990009437443 ) ) ;
#78104=CARTESIAN_POINT ( 'NONE',  ( 3.349194028415048763, -277.5989106332669962, -335.4293566858443114 ) ) ;
#78105=CARTESIAN_POINT ( 'NONE',  ( -103.0629969284240985, -277.8640761644923032, -230.9042351043891870 ) ) ;
#78106=CARTESIAN_POINT ( 'NONE',  ( -49.18953983233350158, -154.2942235963202791, -362.3100455858933060 ) ) ;
#78107=CARTESIAN_POINT ( 'NONE',  ( -32.70881697004364241, -275.0504157368431493, -193.7232294712062810 ) ) ;
#78110=CARTESIAN_POINT ( 'NONE',  ( -73.02176949901455316, -299.0143876308192148, -202.7339417031545281 ) ) ;
#78111=CARTESIAN_POINT ( 'NONE',  ( 35.77081079830085031, -289.8376638359844719, -253.6410175316879361 ) ) ;
#78114=CARTESIAN_POINT ( 'NONE',  ( 29.71334334767416507, -289.0303694817180258, -300.1156040278231103 ) ) ;
#78115=CARTESIAN_POINT ( 'NONE',  ( -105.7763437893944456, -286.7416523193910507, -237.3357707742747778 ) ) ;
#78117=CARTESIAN_POINT ( 'NONE',  ( -21.11476984719934080, -288.1869865413264620, -341.6393011909145798 ) ) ;
#78118=CARTESIAN_POINT ( 'NONE',  ( -66.55869265611643470, -282.9323418135126076, -341.5503888361544682 ) ) ;
#78119=CARTESIAN_POINT ( 'NONE',  ( 17.67262830335883450, -279.2559124369163328, -221.1690039466874680 ) ) ;
#78120=CARTESIAN_POINT ( 'NONE',  ( -1.612341663451327678, -288.3910328146881170, -205.2321168238686937 ) ) ;
#78121=CARTESIAN_POINT ( 'NONE',  ( 27.07418708481774416, -279.5472425279842241, -234.5658497833289005 ) ) ;
#78122=CARTESIAN_POINT ( 'NONE',  ( -64.49990146468725527, -278.7292768637358336, -338.7062659103573310 ) ) ;
#78123=CARTESIAN_POINT ( 'NONE',  ( 35.16795938795580412, -276.1679627353783530, -279.7280099715379151 ) ) ;
#78124=CARTESIAN_POINT ( 'NONE',  ( 30.00623854018101611, -286.8229709056450361, -306.9722039344758286 ) ) ;
#78125=CARTESIAN_POINT ( 'NONE',  ( -27.38287775629013154, -283.7316426767608277, -346.6047914931318701 ) ) ;
#78126=CARTESIAN_POINT ( 'NONE',  ( -102.8623873487384088, -284.5169425481083749, -310.6918314558797078 ) ) ;
#78127=CARTESIAN_POINT ( 'NONE',  ( -10.97378853559589551, -282.8654076314809913, -338.4862295860845620 ) ) ;
#78131=CARTESIAN_POINT ( 'NONE',  ( 26.41834574880639863, -289.9592940477430147, -311.3841986868908407 ) ) ;
#78132=CARTESIAN_POINT ( 'NONE',  ( -81.63118595850768600, -290.1478534872501882, -207.9773082523015546 ) ) ;
#78133=CARTESIAN_POINT ( 'NONE',  ( -110.4226823353708937, -271.6829154849941119, -264.8839556211831905 ) ) ;
#78134=CARTESIAN_POINT ( 'NONE',  ( 37.96907782122586639, -293.0953925575020094, -285.9045896564433633 ) ) ;
#78135=CARTESIAN_POINT ( 'NONE',  ( -78.57826584841215833, -288.0980639559382439, -331.4983610439551853 ) ) ;
#78136=CARTESIAN_POINT ( 'NONE',  ( -5.586818723188489599, -290.7154999873113184, -203.4920638445140924 ) ) ;
#78137=CARTESIAN_POINT ( 'NONE',  ( -107.3260747433741500, -291.4635883352420365, -292.6496351781394196 ) ) ;
#78138=CARTESIAN_POINT ( 'NONE',  ( 31.03373250439201669, -301.4082689599840705, -195.3320873922940848 ) ) ;
#78139=CARTESIAN_POINT ( 'NONE',  ( -72.22056698076656289, -291.5136513959164404, -336.7717638204637751 ) ) ;
#78140=CARTESIAN_POINT ( 'NONE',  ( -95.15213559790508668, -289.2139908476052028, -222.2997750956995731 ) ) ;
#78141=CARTESIAN_POINT ( 'NONE',  ( -111.1497079133605297, -292.3803911499525157, -283.7507008984343315 ) ) ;
#78142=CARTESIAN_POINT ( 'NONE',  ( -27.81778322067169285, -287.1173217162890410, -197.7477345432518803 ) ) ;
#78143=CARTESIAN_POINT ( 'NONE',  ( 18.04707330162870349, -294.8440685000667827, -219.5466298389553685 ) ) ;
#78146=CARTESIAN_POINT ( 'NONE',  ( -31.41511807427017899, -276.1065096258465132, -195.2263364042563865 ) ) ;
#78147=CARTESIAN_POINT ( 'NONE',  ( -110.1958620557682735, -295.4411499741268585, -294.7830325296898195 ) ) ;
#78148=CARTESIAN_POINT ( 'NONE',  ( -35.34077346015080678, -272.3174319252889859, -196.3621547258715907 ) ) ;
#78149=CARTESIAN_POINT ( 'NONE',  ( -106.6166514506029159, -276.2747047338826860, -297.6062150647823614 ) ) ;
#78150=CARTESIAN_POINT ( 'NONE',  ( -34.47241943930104924, -299.4039840146938900, -196.8673052391749820 ) ) ;
#78151=CARTESIAN_POINT ( 'NONE',  ( -15.92497645602875700, -272.8984603680809755, -196.9581903346149829 ) ) ;
#78152=CARTESIAN_POINT ( 'NONE',  ( -95.22576251495287636, -297.3417654636216980, -315.8013010876480280 ) ) ;
#78154=CARTESIAN_POINT ( 'NONE',  ( -110.4023911443710517, -297.3044599074138432, -274.2000181807960644 ) ) ;
#78156=CARTESIAN_POINT ( 'NONE',  ( 1.906320906490790223, -284.5947088680614456, -206.0338325817769487 ) ) ;
#78157=CARTESIAN_POINT ( 'NONE',  ( -72.84688197322741132, -297.5677205883679335, -206.5772480612146182 ) ) ;
#78158=CARTESIAN_POINT ( 'NONE',  ( 2.741011375799959460, -286.5742817885151794, -204.6163369083437544 ) ) ;
#78159=CARTESIAN_POINT ( 'NONE',  ( -57.28951361561180988, -288.9693248741229468, -344.7655802980067392 ) ) ;
#78160=CARTESIAN_POINT ( 'NONE',  ( -110.9982694717852780, -298.7360770413811792, -254.3911565861511974 ) ) ;
#78161=CARTESIAN_POINT ( 'NONE',  ( -56.29155764638935011, -293.2965588898631495, -342.8090991580810396 ) ) ;
#78162=CARTESIAN_POINT ( 'NONE',  ( -56.50647530761765580, -279.0085380875518126, -195.8960865851302344 ) ) ;
#78163=CARTESIAN_POINT ( 'NONE',  ( 35.77081079830085031, -285.2666405000204577, -287.0812184334320705 ) ) ;
#78165=CARTESIAN_POINT ( 'NONE',  ( -68.94276687916048729, -288.2721729156947958, -336.6068958587171664 ) ) ;
#78167=CARTESIAN_POINT ( 'NONE',  ( -61.93421492268576145, -287.3716847480724823, -341.2145502469942357 ) ) ;
#78168=CARTESIAN_POINT ( 'NONE',  ( -39.20877240894571258, -299.6284989585577705, -196.5721919568737235 ) ) ;
#78169=CARTESIAN_POINT ( 'NONE',  ( 25.78351116305544011, -282.4040907476954771, -227.2128857121682586 ) ) ;
#78170=CARTESIAN_POINT ( 'NONE',  ( -100.2689438469268310, -294.0142056378176676, -311.9111575173043320 ) ) ;
#78171=CARTESIAN_POINT ( 'NONE',  ( 32.23131939602069451, -281.8471831943485313, -292.6299335906476813 ) ) ;
#78172=CARTESIAN_POINT ( 'NONE',  ( -113.3898825005471451, -296.8708226820280629, -258.2080291540393659 ) ) ;
#78173=CARTESIAN_POINT ( 'NONE',  ( -110.1685606238186210, -274.1202508383929626, -259.4470971184537120 ) ) ;
#78175=CARTESIAN_POINT ( 'NONE',  ( 35.91759642342782399, -283.7593415629847868, -286.4852652283802854 ) ) ;
#78176=CARTESIAN_POINT ( 'NONE',  ( -104.1561834864384508, -295.2067863679745869, -300.4723459569428314 ) ) ;
#78178=CARTESIAN_POINT ( 'NONE',  ( -32.00346527606124170, -284.9643559479886221, -344.8147952057261136 ) ) ;
#78180=CARTESIAN_POINT ( 'NONE',  ( 10.59707575819633618, -285.9094976428776818, -330.5268031993606428 ) ) ;
#78181=CARTESIAN_POINT ( 'NONE',  ( -4.074031739948677178, -275.8217601209036616, -339.6390031621251069 ) ) ;
#78182=CARTESIAN_POINT ( 'NONE',  ( -36.20400071169095924, -291.9000928814721192, -197.3575075417269318 ) ) ;
#78183=CARTESIAN_POINT ( 'NONE',  ( 35.24672098506439966, -282.9061459568919190, -257.6477834972278060 ) ) ;
#78184=CARTESIAN_POINT ( 'NONE',  ( 32.86545046033224793, -277.4507883913867090, -293.1074676097956058 ) ) ;
#78185=CARTESIAN_POINT ( 'NONE',  ( -109.6611063110171074, -285.6642053532696650, -295.0291090164496381 ) ) ;
#78186=CARTESIAN_POINT ( 'NONE',  ( -76.35109088460164628, -282.3809962773257212, -332.5935568054922555 ) ) ;
#78187=CARTESIAN_POINT ( 'NONE',  ( -95.50732103470559764, -281.2045895960123403, -223.0138773276377719 ) ) ;
#78188=CARTESIAN_POINT ( 'NONE',  ( -110.1025574160018579, -273.0364890683796375, -245.1647362735621414 ) ) ;
#78189=CARTESIAN_POINT ( 'NONE',  ( 33.01890935381643288, -275.7846940342395783, -301.6402586008851472 ) ) ;
#78190=CARTESIAN_POINT ( 'NONE',  ( 17.23113993169376101, -296.1858419071984940, -320.9883767091038749 ) ) ;
#78194=CARTESIAN_POINT ( 'NONE',  ( -112.8871706354899516, -294.7732105220253516, -263.9509943620176955 ) ) ;
#78195=CARTESIAN_POINT ( 'NONE',  ( -6.256133189139672979, -276.1400287222732572, -336.4935480826406433 ) ) ;
#78196=CARTESIAN_POINT ( 'NONE',  ( 12.95351572872406365, -295.8852534934060259, -327.8167220553053767 ) ) ;
#78197=CARTESIAN_POINT ( 'NONE',  ( 30.55751651418675507, -295.2171216475704796, -305.8252561628572721 ) ) ;
#78198=CARTESIAN_POINT ( 'NONE',  ( -7.463671678042305579, -290.6598054510139946, -339.0265230571637289 ) ) ;
#78199=CARTESIAN_POINT ( 'NONE',  ( -73.75584774849309611, -275.5365553449037748, -335.7519926407345565 ) ) ;
#78200=CARTESIAN_POINT ( 'NONE',  ( -106.5987690837830684, -280.1143944106486288, -297.6516400629935220 ) ) ;
#78201=CARTESIAN_POINT ( 'NONE',  ( -109.7045088548589433, -294.4054011891456639, -287.8774202178561268 ) ) ;
#78202=CARTESIAN_POINT ( 'NONE',  ( 36.46869706612780249, -283.1945915462823677, -253.2065130481381345 ) ) ;
#78203=CARTESIAN_POINT ( 'NONE',  ( -77.20566991804004431, -284.4245870164913867, -208.7778095031564476 ) ) ;
#78204=CARTESIAN_POINT ( 'NONE',  ( -111.5753029650709465, -274.4291645131854693, -270.3850168459313181 ) ) ;
#78206=CARTESIAN_POINT ( 'NONE',  ( -71.18425261407487881, -285.2591111901812155, -205.6558699104188292 ) ) ;
#78208=CARTESIAN_POINT ( 'NONE',  ( 39.10248958358808125, -282.5546423019979443, -264.2147069624708706 ) ) ;
#78209=CARTESIAN_POINT ( 'NONE',  ( -113.2083300039566467, -283.2091657554186099, -281.3317456748765721 ) ) ;
#78210=CARTESIAN_POINT ( 'NONE',  ( -108.4340002377611683, -279.1244606192580022, -299.3215233232049854 ) ) ;
#78212=CARTESIAN_POINT ( 'NONE',  ( -79.82397299963848525, -279.1350294293844740, -333.8121289196917019 ) ) ;
#78213=CARTESIAN_POINT ( 'NONE',  ( -28.24530500278205380, -280.8159766702625575, -193.9494060382646126 ) ) ;
#78214=CARTESIAN_POINT ( 'NONE',  ( 27.36219212280433055, -272.6237833571633473, -239.2376011013261916 ) ) ;
#78215=CARTESIAN_POINT ( 'NONE',  ( 122.8483417650791836, 148.9427304151107307, -263.5502861110473418 ) ) ;
#78216=ORIENTED_EDGE ( 'NONE', *, *, #80097, .T. ) ;
#78217=CARTESIAN_POINT ( 'NONE',  ( -3.292708276216301577, -276.5029539112508701, -203.7081979764361392 ) ) ;
#78218=CARTESIAN_POINT ( 'NONE',  ( 202.8071895515903122, 295.9636489450776367, -54.00000000004035883 ) ) ;
#78219=CARTESIAN_POINT ( 'NONE',  ( -34.21985529895107447, -278.1116752371696634, -195.7687982677718423 ) ) ;
#78220=CARTESIAN_POINT ( 'NONE',  ( 23.15468906069257216, -294.6911167974343471, -224.3597084903977077 ) ) ;
#78221=CARTESIAN_POINT ( 'NONE',  ( 3.867018498677363247, -293.8293822646695048, -330.7410333277059635 ) ) ;
#78222=CARTESIAN_POINT ( 'NONE',  ( -65.43040447464409226, -288.9171951892036532, -342.0452869295789924 ) ) ;
#78224=CARTESIAN_POINT ( 'NONE',  ( -30.66068886033499652, -293.5439739987444341, -346.4792523598452476 ) ) ;
#78225=CARTESIAN_POINT ( 'NONE',  ( -98.00201650591019131, -283.5315760617929755, -228.3058677575226625 ) ) ;
#78226=CARTESIAN_POINT ( 'NONE',  ( -30.71999500373535241, -293.9971708917041155, -196.4218286878305548 ) ) ;
#78227=CARTESIAN_POINT ( 'NONE',  ( -1.835491417002458325, -285.0110408916730194, -205.7281883333272106 ) ) ;
#78228=CARTESIAN_POINT ( 'NONE',  ( -61.68236061479817778, -284.6902125115734066, -339.7600452678200895 ) ) ;
#78230=CARTESIAN_POINT ( 'NONE',  ( -79.47531798111366186, -292.4396946352862869, -206.1292101712163856 ) ) ;
#78231=CARTESIAN_POINT ( 'NONE',  ( -33.48671308066791141, -283.4947028727016800, -343.3334675316916105 ) ) ;
#78232=CARTESIAN_POINT ( 'NONE',  ( 35.98509963879727280, -292.6287501404636373, -292.7034723565416243 ) ) ;
#78233=CARTESIAN_POINT ( 'NONE',  ( -54.45568091545072065, -290.0693200335015263, -345.3241275155259018 ) ) ;
#78234=CARTESIAN_POINT ( 'NONE',  ( -112.5038811090080912, -290.8387653768328391, -286.7980718894850725 ) ) ;
#78235=CARTESIAN_POINT ( 'NONE',  ( 35.63009059669786893, -287.7636400287147467, -273.7577124809947122 ) ) ;
#78237=FACE_OUTER_BOUND ( 'NONE', #55861, .T. ) ;
#78238=CARTESIAN_POINT ( 'NONE',  ( -109.6142948817539633, -298.1216896178034403, -293.1416382998448285 ) ) ;
#78239=CARTESIAN_POINT ( 'NONE',  ( -82.66487049059166736, -296.1323356984701718, -208.6583963620937539 ) ) ;
#78241=CARTESIAN_POINT ( 'NONE',  ( -108.0505578942962046, -277.3598136360681110, -289.4311437306490120 ) ) ;
#78242=CARTESIAN_POINT ( 'NONE',  ( -58.09898027320685543, -273.2987220833773563, -196.2202324819549517 ) ) ;
#78243=CARTESIAN_POINT ( 'NONE',  ( -99.32687365041907412, -294.4845456379242137, -310.3112039782097895 ) ) ;
#78244=CARTESIAN_POINT ( 'NONE',  ( 33.49263129951447837, -277.5930543212922998, -291.8636966324963851 ) ) ;
#78245=CARTESIAN_POINT ( 'NONE',  ( -37.80669735810238308, -296.2861075207721342, -196.3492419481402749 ) ) ;
#78246=CARTESIAN_POINT ( 'NONE',  ( -28.83480362977233824, -296.1471247591911720, -343.3148325497661517 ) ) ;
#78247=CARTESIAN_POINT ( 'NONE',  ( -12.89224436125023665, -295.8065999431065052, -339.5264730276013552 ) ) ;
#78248=CARTESIAN_POINT ( 'NONE',  ( -53.10365836173552623, -296.8509630773195909, -344.9670938096699615 ) ) ;
#78249=CARTESIAN_POINT ( 'NONE',  ( -86.24960189229837226, -295.3757364917250356, -213.2132306156502750 ) ) ;
#78250=CARTESIAN_POINT ( 'NONE',  ( -65.37370893771648639, -292.3272120712665583, -202.8338881731086190 ) ) ;
#78251=CARTESIAN_POINT ( 'NONE',  ( 7.906247026854799742, -299.2561368632369749, -193.4581864202968688 ) ) ;
#78252=CARTESIAN_POINT ( 'NONE',  ( -91.03501290151477576, -288.4078789402160510, -320.7585411176893331 ) ) ;
#78253=CARTESIAN_POINT ( 'NONE',  ( -66.61667398526682859, -275.6688505030992928, -201.3105817330240654 ) ) ;
#78254=CARTESIAN_POINT ( 'NONE',  ( -66.20995228424645518, -274.1766140077583600, -199.0297031343532694 ) ) ;
#78255=CARTESIAN_POINT ( 'NONE',  ( -72.86087804014364622, -297.9009479429373073, -206.5608398698246049 ) ) ;
#78256=CARTESIAN_POINT ( 'NONE',  ( -66.74443605542816726, -281.6487294461595638, -200.9789450227856094 ) ) ;
#78257=CARTESIAN_POINT ( 'NONE',  ( -11.65902343234288097, -279.0644222654100872, -198.2381707162253690 ) ) ;
#78259=CARTESIAN_POINT ( 'NONE',  ( -76.71284650256086479, -282.9128417912821760, -336.4775758886877952 ) ) ;
#78260=CARTESIAN_POINT ( 'NONE',  ( 38.08077018398219593, -275.0884878916513117, -285.3532412132651643 ) ) ;
#78261=CARTESIAN_POINT ( 'NONE',  ( 31.30966784710482997, -279.5219981305814372, -237.1726039575034122 ) ) ;
#78262=CARTESIAN_POINT ( 'NONE',  ( 16.49497035111065202, -280.2894872588807971, -322.8915533308707495 ) ) ;
#78263=CARTESIAN_POINT ( 'NONE',  ( -35.35638404869035867, -272.6522467003142083, -196.7860660831684640 ) ) ;
#78264=CARTESIAN_POINT ( 'NONE',  ( 31.37081170764443527, -277.1573261644568333, -240.1737162067874749 ) ) ;
#78267=CARTESIAN_POINT ( 'NONE',  ( -98.26636462649079817, -295.4043386109883613, -224.9284058695760109 ) ) ;
#78268=CARTESIAN_POINT ( 'NONE',  ( -14.34391950530947746, -290.3688540135494804, -198.5462537631774183 ) ) ;
#78269=CARTESIAN_POINT ( 'NONE',  ( 1.700100917900669639, -292.5587675933670084, -203.9319858678950368 ) ) ;
#78270=CARTESIAN_POINT ( 'NONE',  ( 36.68209423794102975, -277.3840819315672661, -257.2299041075381183 ) ) ;
#78271=CARTESIAN_POINT ( 'NONE',  ( -46.39563600217162076, -271.9370851214541744, -195.9096109961765819 ) ) ;
#78273=CARTESIAN_POINT ( 'NONE',  ( 34.25268226494973334, -283.7842335365593840, -294.6808344674290083 ) ) ;
#78275=CARTESIAN_POINT ( 'NONE',  ( -111.8967894818025854, -282.6625610866086618, -261.7495260186613564 ) ) ;
#78277=CARTESIAN_POINT ( 'NONE',  ( -55.91854954511688902, -294.0915156814653528, -341.4210509019096094 ) ) ;
#78278=CARTESIAN_POINT ( 'NONE',  ( 21.33123772657210893, -285.0618616834468639, -224.8819815898654042 ) ) ;
#78280=CARTESIAN_POINT ( 'NONE',  ( 13.69777801911289394, -292.3372727896691003, -325.3865505291607292 ) ) ;
#78281=CARTESIAN_POINT ( 'NONE',  ( -49.99774993565495862, -281.6905643934345562, -345.6643079940985217 ) ) ;
#78282=CARTESIAN_POINT ( 'NONE',  ( -32.93538861181966837, -281.7087219086758410, -196.6927744773726943 ) ) ;
#78283=CARTESIAN_POINT ( 'NONE',  ( -95.52507491415474306, -286.4336857164828416, -220.4548070453019193 ) ) ;
#78284=CARTESIAN_POINT ( 'NONE',  ( 34.37879508655905170, -279.4693874069580488, -245.1011474304457352 ) ) ;
#78285=CARTESIAN_POINT ( 'NONE',  ( 32.27359270981354200, -287.2604090777331862, -248.3485840590310261 ) ) ;
#78286=CARTESIAN_POINT ( 'NONE',  ( -98.12537369434022594, -279.4049043940268007, -311.8426794918250380 ) ) ;
#78287=CARTESIAN_POINT ( 'NONE',  ( -89.19306452860043066, -278.6072687886634185, -322.0473644619289644 ) ) ;
#78288=CARTESIAN_POINT ( 'NONE',  ( -51.88116316873244216, -287.8470255392998638, -196.3686488436300408 ) ) ;
#78290=CARTESIAN_POINT ( 'NONE',  ( -101.5485180013057374, -296.9448233496169678, -227.8343504451467254 ) ) ;
#78291=CARTESIAN_POINT ( 'NONE',  ( 22.50703440647753339, -290.1443688299032715, -314.9916680717385020 ) ) ;
#78293=CARTESIAN_POINT ( 'NONE',  ( -88.52914483777347243, -287.9090924074130839, -206.2264541496106460 ) ) ;
#78295=CARTESIAN_POINT ( 'NONE',  ( -41.07559082729378019, -272.0052366226703384, -195.2362280283337270 ) ) ;
#78296=CARTESIAN_POINT ( 'NONE',  ( 8.409404898755894919, -292.8372702006462305, -331.2977802006754473 ) ) ;
#78297=CARTESIAN_POINT ( 'NONE',  ( -109.2284136122852942, -272.0791603529684153, -256.8167345609106178 ) ) ;
#78298=CARTESIAN_POINT ( 'NONE',  ( 34.96820303596955881, -289.2588488277343686, -284.6386020409750017 ) ) ;
#78299=CARTESIAN_POINT ( 'NONE',  ( -16.65973667170447925, -282.0831840653772247, -199.2961449017545874 ) ) ;
#78300=CARTESIAN_POINT ( 'NONE',  ( -57.12073960555999719, -290.7275953252116665, -344.2222733945458799 ) ) ;
#78301=CARTESIAN_POINT ( 'NONE',  ( -74.17510388940996791, -290.8462840822272710, -337.4327558389133515 ) ) ;
#78302=CARTESIAN_POINT ( 'NONE',  ( -109.2804093825592275, -286.8275520544906385, -248.9717581267117055 ) ) ;
#78303=CARTESIAN_POINT ( 'NONE',  ( -19.75828574208869526, -280.4387327722728855, -195.3408655458659666 ) ) ;
#78304=CARTESIAN_POINT ( 'NONE',  ( -6.409975722179727775, -292.7288920642370726, -339.2998054251737017 ) ) ;
#78305=CARTESIAN_POINT ( 'NONE',  ( 26.28181498157088569, -280.8123952974474946, -226.8970263228519855 ) ) ;
#78306=CARTESIAN_POINT ( 'NONE',  ( 35.03278656305512584, -277.1976479175255008, -253.7877331182183411 ) ) ;
#78307=CARTESIAN_POINT ( 'NONE',  ( -106.6662871844225293, -299.4805209788416391, -237.0123917617630980 ) ) ;
#78308=CARTESIAN_POINT ( 'NONE',  ( 23.54211671714417875, -274.4049405898031182, -315.8268728129942247 ) ) ;
#78310=CARTESIAN_POINT ( 'NONE',  ( 7.184788178814246251, -280.1849474899177608, -212.3714581194895175 ) ) ;
#78311=CARTESIAN_POINT ( 'NONE',  ( -25.81449592184696584, -278.1135081855322255, -346.0917741324411168 ) ) ;
#78312=CARTESIAN_POINT ( 'NONE',  ( -6.336058425474879741, -275.7834175514993831, -203.7285909245110247 ) ) ;
#78313=CARTESIAN_POINT ( 'NONE',  ( -1.070120186143436625, -285.5803442769611706, -202.7061647127713684 ) ) ;
#78314=CARTESIAN_POINT ( 'NONE',  ( -106.9785084891391023, -291.9829201981611391, -295.4347881104945372 ) ) ;
#78315=CARTESIAN_POINT ( 'NONE',  ( -60.64604339787312881, -275.3550378565459482, -197.7571250308804451 ) ) ;
#78316=CARTESIAN_POINT ( 'NONE',  ( -103.8094469705283842, -274.3637462301140317, -232.3689197104448283 ) ) ;
#78318=CARTESIAN_POINT ( 'NONE',  ( -109.3604362198488502, -298.2901384300380414, -290.6916388824978981 ) ) ;
#78319=CARTESIAN_POINT ( 'NONE',  ( -38.94937919989016706, -281.0721757532335232, -345.1899886907590371 ) ) ;
#78320=CARTESIAN_POINT ( 'NONE',  ( -92.79390621262160721, -290.9507028680513940, -216.8924315482295242 ) ) ;
#78321=CARTESIAN_POINT ( 'NONE',  ( 24.42727591624192129, -273.0020381159397402, -228.4282720569481455 ) ) ;
#78322=CARTESIAN_POINT ( 'NONE',  ( 7.061050246335325298, -288.2454037619567657, -208.3700882003813604 ) ) ;
#78323=CARTESIAN_POINT ( 'NONE',  ( -69.13929068415136214, -290.5441636556618619, -204.2931938160888876 ) ) ;
#78325=CARTESIAN_POINT ( 'NONE',  ( -111.6935907602036053, -288.9041413973887416, -288.0354051462061875 ) ) ;
#78326=CARTESIAN_POINT ( 'NONE',  ( -95.12852218884312094, -290.8471963740800561, -225.7206578260619665 ) ) ;
#78328=CARTESIAN_POINT ( 'NONE',  ( -1.127709513165200628, -287.6009411039925112, -202.7590514895931619 ) ) ;
#78329=CARTESIAN_POINT ( 'NONE',  ( -100.5990294264053233, -278.3841973351577508, -306.9400203185992950 ) ) ;
#78330=CARTESIAN_POINT ( 'NONE',  ( 1.600581836954556803, -293.4645680352248860, -336.4291979080119290 ) ) ;
#78331=CARTESIAN_POINT ( 'NONE',  ( -114.2250769792311331, -285.2440651346432787, -267.1269796536276431 ) ) ;
#78332=CARTESIAN_POINT ( 'NONE',  ( -112.5035268974379363, -284.6774356220762456, -286.9877258253117702 ) ) ;
#78333=CARTESIAN_POINT ( 'NONE',  ( 5.607951058262628408, -282.7853120791038464, -329.4154569396601460 ) ) ;
#78334=CARTESIAN_POINT ( 'NONE',  ( -63.59754655805116386, -182.8661901358721309, -362.5093420553077976 ) ) ;
#78335=CARTESIAN_POINT ( 'NONE',  ( -32.41727912486597063, -123.7363485282854896, -362.9951886188725894 ) ) ;
#78336=CARTESIAN_POINT ( 'NONE',  ( -112.1542233637230908, -270.3668851746004407, -283.6615718338756551 ) ) ;
#78337=CARTESIAN_POINT ( 'NONE',  ( -74.34624968938332756, -272.7440816174270708, -207.1893234989277914 ) ) ;
#78338=CARTESIAN_POINT ( 'NONE',  ( 29.37303827091535169, -274.0630553738110393, -239.8512678150489137 ) ) ;
#78339=CARTESIAN_POINT ( 'NONE',  ( -72.05188845079854332, -295.0064864794960613, -339.0250075467953934 ) ) ;
#78340=CARTESIAN_POINT ( 'NONE',  ( 203.3290562182569943, 291.9839156117442940, -53.99999999998728129 ) ) ;
#78341=CARTESIAN_POINT ( 'NONE',  ( -1.517488088399022050, -273.2018580692800924, -202.7599041949939931 ) ) ;
#78342=CARTESIAN_POINT ( 'NONE',  ( -110.2634163752252192, -298.5937993823400234, -256.3904709118299934 ) ) ;
#78343=CARTESIAN_POINT ( 'NONE',  ( -44.34335962587524449, -293.0413301273801494, -197.3360970108299455 ) ) ;
#78344=ORIENTED_EDGE ( 'NONE', *, *, #85799, .F. ) ;
#78345=CARTESIAN_POINT ( 'NONE',  ( -87.31819247139647189, -298.3166755962409979, -212.0229436309392668 ) ) ;
#78346=CARTESIAN_POINT ( 'NONE',  ( -18.45155229318037371, -289.2946306705424604, -340.9910173114611212 ) ) ;
#78347=CARTESIAN_POINT ( 'NONE',  ( 33.27222314002835191, -294.7431795583277108, -300.7912860737888536 ) ) ;
#78348=CARTESIAN_POINT ( 'NONE',  ( -47.61714456234479087, -295.6718046058143159, -346.6103287640002577 ) ) ;
#78349=CARTESIAN_POINT ( 'NONE',  ( 30.58634157623776417, -294.0780099583164997, -297.2348242193176020 ) ) ;
#78351=CARTESIAN_POINT ( 'NONE',  ( 17.03597120988462521, -276.7395145957429463, -217.8228770296917105 ) ) ;
#78354=CARTESIAN_POINT ( 'NONE',  ( -106.1177533559898336, -278.5051262261009697, -235.7550713857343112 ) ) ;
#78356=CARTESIAN_POINT ( 'NONE',  ( 33.08297254554128841, -276.2264248726715437, -250.0858929216487923 ) ) ;
#78357=CARTESIAN_POINT ( 'NONE',  ( -27.15485575526050255, -275.9399409156598608, -195.0076471617659877 ) ) ;
#78358=CARTESIAN_POINT ( 'NONE',  ( 30.36609332827191565, -274.0076102129252718, -303.5564886503789808 ) ) ;
#78359=CARTESIAN_POINT ( 'NONE',  ( -69.30959058829047592, -298.2714248764343097, -204.6196040959292191 ) ) ;
#78360=CARTESIAN_POINT ( 'NONE',  ( -68.78546357107944687, -294.0484813987965822, -336.9081459888010386 ) ) ;
#78362=CARTESIAN_POINT ( 'NONE',  ( -96.77390321102514292, -279.7015354658562387, -221.4802143903870899 ) ) ;
#78363=CARTESIAN_POINT ( 'NONE',  ( 33.58703610328374367, -275.9472700432625629, -287.6797706704508641 ) ) ;
#78365=CARTESIAN_POINT ( 'NONE',  ( 26.73394810780187569, -285.6842630779813135, -228.5566974557147262 ) ) ;
#78366=CARTESIAN_POINT ( 'NONE',  ( -67.46667442081138688, -299.6582395621390447, -201.4397465638191420 ) ) ;
#78367=CARTESIAN_POINT ( 'NONE',  ( 82.68044179851318631, -297.0770420877388460, -195.7386261002818912 ) ) ;
#78368=CARTESIAN_POINT ( 'NONE',  ( 35.81655398972591087, -286.7583535030299799, -271.0478354302956063 ) ) ;
#78369=CARTESIAN_POINT ( 'NONE',  ( 19.63028343106945428, -279.1309812026076997, -223.0956244082971125 ) ) ;
#78370=CARTESIAN_POINT ( 'NONE',  ( -65.02104947398494517, -278.2580079355589646, -202.1758663696145675 ) ) ;
#78371=CARTESIAN_POINT ( 'NONE',  ( -86.82248143355772640, -287.3644923948191376, -213.9312115247869315 ) ) ;
#78372=CARTESIAN_POINT ( 'NONE',  ( -8.568951285032019527, -277.8720777042691452, -337.8970240043456101 ) ) ;
#78374=CARTESIAN_POINT ( 'NONE',  ( -41.35365668423214913, -275.3418465024450370, -346.2548370054150837 ) ) ;
#78375=CARTESIAN_POINT ( 'NONE',  ( -38.09171799484808218, -274.6939233269887950, -197.2630322226893611 ) ) ;
#78376=CARTESIAN_POINT ( 'NONE',  ( 34.41771835781664635, -283.2643670656914878, -247.9867065829535306 ) ) ;
#78378=CARTESIAN_POINT ( 'NONE',  ( 15.69299422997897153, -290.2292460827072205, -324.2542994614541954 ) ) ;
#78379=CARTESIAN_POINT ( 'NONE',  ( -8.888675440074152334, -290.4241454990054763, -200.9541106807363064 ) ) ;
#78381=CARTESIAN_POINT ( 'NONE',  ( 28.30927743145671727, -273.7916668127161870, -237.3279131416217353 ) ) ;
#78382=CARTESIAN_POINT ( 'NONE',  ( 34.97337904310720802, -291.9099984919495796, -287.1918667519220776 ) ) ;
#78383=CARTESIAN_POINT ( 'NONE',  ( -111.8441652935849646, -278.1196860901031300, -270.4320060261264871 ) ) ;
#78385=CARTESIAN_POINT ( 'NONE',  ( -98.48529726871387879, -288.4189354325264958, -316.0354243202887119 ) ) ;
#78386=CARTESIAN_POINT ( 'NONE',  ( -74.17862599039634119, -285.1502030596065538, -334.3683977373329412 ) ) ;
#78387=CARTESIAN_POINT ( 'NONE',  ( 34.97637758395062235, -286.0892622408953230, -293.6864186126551886 ) ) ;
#78388=CARTESIAN_POINT ( 'NONE',  ( -99.51925121296332577, -285.4366913320662320, -309.8179703291999658 ) ) ;
#78389=CARTESIAN_POINT ( 'NONE',  ( -51.03812470570034066, -284.0343867308039307, -342.2808091758216733 ) ) ;
#78390=CARTESIAN_POINT ( 'NONE',  ( -35.03654083359199944, -294.0608247401532367, -195.0283106696795983 ) ) ;
#78391=CARTESIAN_POINT ( 'NONE',  ( 36.81038724188080380, -273.4469698837517626, -255.8427799423238014 ) ) ;
#78392=CARTESIAN_POINT ( 'NONE',  ( 22.62720205646445848, -276.5326587223444221, -318.6466053410275663 ) ) ;
#78393=CARTESIAN_POINT ( 'NONE',  ( -111.1638028333777868, -288.4266546160624785, -286.4735775844918635 ) ) ;
#78394=CARTESIAN_POINT ( 'NONE',  ( -98.80342328284632458, -277.9342014865476926, -316.7665546254544893 ) ) ;
#78395=CARTESIAN_POINT ( 'NONE',  ( -42.47829642095573632, -297.0971599397786918, -344.8289780431859413 ) ) ;
#78398=CARTESIAN_POINT ( 'NONE',  ( -78.66766804204782204, -282.3066913607690935, -331.1345320139957380 ) ) ;
#78400=CARTESIAN_POINT ( 'NONE',  ( -2.053338970258056229, -278.5192938388750008, -204.1815726689978021 ) ) ;
#78403=CARTESIAN_POINT ( 'NONE',  ( 9.103795711878566621, -273.1567691800516968, -209.8175496446503701 ) ) ;
#78404=CARTESIAN_POINT ( 'NONE',  ( -11.22536265483237372, -276.0511823895362227, -338.6387100988942507 ) ) ;
#78405=CARTESIAN_POINT ( 'NONE',  ( 10.75856280437803214, -295.8928824573421252, -326.1918662891938538 ) ) ;
#78406=CARTESIAN_POINT ( 'NONE',  ( 37.37945845847486481, -280.2549802172915179, -253.0337193628718353 ) ) ;
#78407=CARTESIAN_POINT ( 'NONE',  ( -15.51129814104582216, -295.7039670232302910, -340.3204145593449539 ) ) ;
#78408=CARTESIAN_POINT ( 'NONE',  ( -96.12171209824758478, -297.2041448875631318, -319.3529893802767674 ) ) ;
#78409=CARTESIAN_POINT ( 'NONE',  ( -96.29592946883931859, -272.8230558558606731, -227.1901537869062224 ) ) ;
#78410=CARTESIAN_POINT ( 'NONE',  ( -87.27917837666056755, -293.3566860727104881, -214.3336309366040950 ) ) ;
#78411=CARTESIAN_POINT ( 'NONE',  ( -49.34682206839899976, -286.0699846215512139, -194.2490027569031383 ) ) ;
#78412=CARTESIAN_POINT ( 'NONE',  ( -8.144324461542206350, -272.5699349044903101, -200.3924827513508546 ) ) ;
#78413=CARTESIAN_POINT ( 'NONE',  ( 25.54633227888296432, -286.7972556030635474, -225.9075912452445323 ) ) ;
#78414=CARTESIAN_POINT ( 'NONE',  ( -86.58781622024113744, -281.3436857260083457, -214.2659591026491057 ) ) ;
#78415=CARTESIAN_POINT ( 'NONE',  ( 0.2998550268531107732, -285.6252057537514588, -207.4806428895656722 ) ) ;
#78417=CARTESIAN_POINT ( 'NONE',  ( -48.59473957666993016, -287.1951287104843118, -344.5646564750267089 ) ) ;
#78418=CARTESIAN_POINT ( 'NONE',  ( -110.2140130185358942, -271.2396475792842807, -270.3444066551136871 ) ) ;
#78419=CARTESIAN_POINT ( 'NONE',  ( 35.05799769567690305, -286.9256033758499598, -260.1795142919913815 ) ) ;
#78420=CARTESIAN_POINT ( 'NONE',  ( -8.117325910327814142, -283.6200023080649544, -341.4016855523141771 ) ) ;
#78421=CARTESIAN_POINT ( 'NONE',  ( -66.91369441533387885, -290.7326943542555000, -199.5210349282357640 ) ) ;
#78422=CARTESIAN_POINT ( 'NONE',  ( -96.21251145214854716, -280.8091371125991600, -221.9603711676448654 ) ) ;
#78423=CARTESIAN_POINT ( 'NONE',  ( -111.2589409935327609, -280.1166075648310425, -250.5737354612289778 ) ) ;
#78424=CARTESIAN_POINT ( 'NONE',  ( 25.55795177190707079, -281.8955526958179121, -307.5100733637838744 ) ) ;
#78425=CARTESIAN_POINT ( 'NONE',  ( 6.320955576305673063, -276.6447947840239294, -209.3168402642163244 ) ) ;
#78426=CARTESIAN_POINT ( 'NONE',  ( 1.769434916572098615, -294.5440652500597594, -336.6884812312139843 ) ) ;
#78427=CARTESIAN_POINT ( 'NONE',  ( -18.07268976553725892, -286.8227891367428697, -342.5297369036424016 ) ) ;
#78429=CARTESIAN_POINT ( 'NONE',  ( -110.0409435198949240, -295.6014632553917068, -260.5417629004472246 ) ) ;
#78432=CARTESIAN_POINT ( 'NONE',  ( -40.26694038014439769, -285.0093664185279749, -344.7436237853778493 ) ) ;
#78433=CARTESIAN_POINT ( 'NONE',  ( -47.80025952003029488, -294.8553954343872761, -342.6807050971036119 ) ) ;
#78435=CARTESIAN_POINT ( 'NONE',  ( 38.01892542963208399, -294.4532349136481457, -256.1390004877245019 ) ) ;
#78436=CARTESIAN_POINT ( 'NONE',  ( -88.96040021043248203, -284.4523281539379695, -322.1951046163125625 ) ) ;
#78437=CARTESIAN_POINT ( 'NONE',  ( 7.108535864358120016, -273.6996941862225867, -207.7099614268474284 ) ) ;
#78438=CARTESIAN_POINT ( 'NONE',  ( -100.5920300223631330, -290.6252149670721678, -314.0956415870195997 ) ) ;
#78439=CARTESIAN_POINT ( 'NONE',  ( -58.17029636089915812, -281.4579371267788588, -343.2612872958006847 ) ) ;
#78440=CARTESIAN_POINT ( 'NONE',  ( -96.56532263054504028, -291.5470550255757303, -221.1644630560952578 ) ) ;
#78441=CARTESIAN_POINT ( 'NONE',  ( 34.30572813080871697, -288.0721999624807381, -284.5230614834006246 ) ) ;
#78444=CARTESIAN_POINT ( 'NONE',  ( -102.0040017515520532, -254.2189882600752640, -324.0990601116661765 ) ) ;
#78445=CARTESIAN_POINT ( 'NONE',  ( 39.58706461736021254, -285.0523547857346784, -270.3937649182068981 ) ) ;
#78447=CARTESIAN_POINT ( 'NONE',  ( -51.87524831574088324, -278.7822462262372483, -198.4551371268680668 ) ) ;
#78448=CARTESIAN_POINT ( 'NONE',  ( -26.99515829319025784, -273.8468557075844956, -194.0273421752997649 ) ) ;
#78449=CARTESIAN_POINT ( 'NONE',  ( -40.55973565844323048, -279.0928470218787538, -345.1380091550995530 ) ) ;
#78450=CARTESIAN_POINT ( 'NONE',  ( -81.45210018623211568, -220.0163494656852947, -350.2350564171413225 ) ) ;
#78451=CARTESIAN_POINT ( 'NONE',  ( 38.28547164587251928, -280.2644431678554042, -281.2761160248477381 ) ) ;
#78452=CARTESIAN_POINT ( 'NONE',  ( 1.946051286740130282, -280.5441342584977633, -333.8905056948813126 ) ) ;
#78453=CARTESIAN_POINT ( 'NONE',  ( -96.57077276360662665, -298.9586978438368305, -222.7597422412592607 ) ) ;
#78454=CARTESIAN_POINT ( 'NONE',  ( 26.28506580502691747, -293.5521184276691997, -234.3465108053729296 ) ) ;
#78456=CARTESIAN_POINT ( 'NONE',  ( -64.23658967843672940, -290.3785769373666312, -201.9522582982607446 ) ) ;
#78457=CARTESIAN_POINT ( 'NONE',  ( -24.18521922064208240, -274.8672001459042349, -194.5427860907640820 ) ) ;
#78458=CARTESIAN_POINT ( 'NONE',  ( -49.95600444325668832, -298.0533782744596465, -198.4592450505566319 ) ) ;
#78463=CARTESIAN_POINT ( 'NONE',  ( 7.319803951760524008, -281.7567131493385091, -212.1627766860408713 ) ) ;
#78464=CARTESIAN_POINT ( 'NONE',  ( -40.98256546537702150, -281.7670953062150829, -194.4487015466088451 ) ) ;
#78465=CARTESIAN_POINT ( 'NONE',  ( -70.33161826673779160, -282.5567461330404058, -335.7591906940342028 ) ) ;
#78466=CARTESIAN_POINT ( 'NONE',  ( -16.59889848231464526, -282.1834426315358542, -199.0827786510282635 ) ) ;
#78467=CARTESIAN_POINT ( 'NONE',  ( 32.75173006594489067, -274.3310413565459385, -293.1123552247106545 ) ) ;
#78470=CARTESIAN_POINT ( 'NONE',  ( -70.22261918109316525, -278.2772412999402150, -339.8233752520499706 ) ) ;
#78474=CARTESIAN_POINT ( 'NONE',  ( -112.5131042436098028, -286.6081755116678664, -264.4039219905544655 ) ) ;
#78475=CARTESIAN_POINT ( 'NONE',  ( 34.48095159329980675, -292.9327012606881908, -284.2933980217973726 ) ) ;
#78476=CARTESIAN_POINT ( 'NONE',  ( 36.68403091330414156, -287.1625547339869513, -291.2301462495102555 ) ) ;
#78477=CARTESIAN_POINT ( 'NONE',  ( -79.87352801256264456, -283.7083829713150749, -209.7257957932574470 ) ) ;
#78478=CARTESIAN_POINT ( 'NONE',  ( -107.9148938436018170, -283.4026722296071057, -249.3326970086081360 ) ) ;
#78479=CARTESIAN_POINT ( 'NONE',  ( -98.96665030307347877, -288.2305241148876576, -311.3761454465097245 ) ) ;
#78481=CARTESIAN_POINT ( 'NONE',  ( -13.38534140587776733, -283.9392215877786043, -339.7924165430966355 ) ) ;
#78482=CARTESIAN_POINT ( 'NONE',  ( 29.48023259841298582, -273.1017076613928793, -236.3048417269511106 ) ) ;
#78483=CARTESIAN_POINT ( 'NONE',  ( -109.2158436419237546, -283.2746638471179494, -245.0520700225553696 ) ) ;
#78484=CARTESIAN_POINT ( 'NONE',  ( -99.94444018351963166, -297.9936164148192006, -311.7575081680385551 ) ) ;
#78485=CARTESIAN_POINT ( 'NONE',  ( -65.17426539874490743, -283.6891656536947153, -200.5234046843481792 ) ) ;
#78486=CARTESIAN_POINT ( 'NONE',  ( -110.5869072513067977, -279.5256099270086452, -267.9123145746898444 ) ) ;
#78487=CARTESIAN_POINT ( 'NONE',  ( 25.58861575695056700, -288.9990628942610442, -229.2538951532462761 ) ) ;
#78490=CARTESIAN_POINT ( 'NONE',  ( 28.21393930871990463, -294.9747986362789902, -232.7875590099642409 ) ) ;
#78491=CARTESIAN_POINT ( 'NONE',  ( -110.2274324427090164, -276.7790754386518302, -252.6786216133278913 ) ) ;
#78492=CARTESIAN_POINT ( 'NONE',  ( -79.49726655252457874, -290.6958910110059264, -206.0552681249102989 ) ) ;
#78493=CARTESIAN_POINT ( 'NONE',  ( -82.86917528380666909, -294.0862573907730848, -328.5097559344705473 ) ) ;
#78494=CARTESIAN_POINT ( 'NONE',  ( -89.81402319500199383, -277.9775472419046878, -218.8312759855063518 ) ) ;
#78495=CARTESIAN_POINT ( 'NONE',  ( -93.99410272325668814, -271.3057950871630624, -222.0525330141317966 ) ) ;
#78496=CARTESIAN_POINT ( 'NONE',  ( -95.51494404148783701, -292.4953847904963595, -225.4487903644360358 ) ) ;
#78497=CARTESIAN_POINT ( 'NONE',  ( 10.59707575819634329, -283.1948066931273615, -210.1954327657594490 ) ) ;
#78498=CARTESIAN_POINT ( 'NONE',  ( -34.89642681218753495, -293.5018399251170536, -346.6285972431149958 ) ) ;
#78499=CARTESIAN_POINT ( 'NONE',  ( -20.93185143611571064, -290.4381658120578891, -342.3135833948044251 ) ) ;
#78500=CARTESIAN_POINT ( 'NONE',  ( 10.49843300442863026, -290.9418648339523088, -211.2570125170873609 ) ) ;
#78501=CARTESIAN_POINT ( 'NONE',  ( -109.5130702540078431, -291.7884607331311599, -284.8014540948812510 ) ) ;
#78503=CARTESIAN_POINT ( 'NONE',  ( -62.86662375479551201, -292.5139747021296444, -201.7966957155939838 ) ) ;
#78505=CARTESIAN_POINT ( 'NONE',  ( -110.8554476210593549, -292.0287250168922810, -248.8265492972847142 ) ) ;
#78506=CARTESIAN_POINT ( 'NONE',  ( 23.75853565688203872, -280.1701052742652109, -314.4870708245243804 ) ) ;
#78507=CARTESIAN_POINT ( 'NONE',  ( 35.53467388016392903, -293.4856031940490766, -265.3163420777694910 ) ) ;
#78508=CARTESIAN_POINT ( 'NONE',  ( 6.184255125203040215, -280.6253157357538157, -206.8434730381110285 ) ) ;
#78509=CARTESIAN_POINT ( 'NONE',  ( 31.05641446366167102, -281.6742719479181005, -305.6802659299880816 ) ) ;
#78510=CARTESIAN_POINT ( 'NONE',  ( 3.558444390643651811, -284.6021483064833433, -207.4947611173977009 ) ) ;
#78511=CARTESIAN_POINT ( 'NONE',  ( 34.14258903376332199, -279.9519642562785862, -290.3826535109857332 ) ) ;
#78513=CARTESIAN_POINT ( 'NONE',  ( -72.64837932770662121, -283.5848898623127639, -204.1338314561199070 ) ) ;
#78515=CARTESIAN_POINT ( 'NONE',  ( -59.08588370616837437, -278.2556155432524179, -197.2181194678722420 ) ) ;
#78516=CARTESIAN_POINT ( 'NONE',  ( -65.75002696594327745, -284.6095061475264174, -199.1117810749830142 ) ) ;
#78517=CARTESIAN_POINT ( 'NONE',  ( -29.98377074073661674, -274.9504960968371279, -197.5705787482251594 ) ) ;
#78519=CARTESIAN_POINT ( 'NONE',  ( -6.959312775711741672, -294.0577942450718183, -203.1052561125959528 ) ) ;
#78520=CARTESIAN_POINT ( 'NONE',  ( 15.60557607635313637, -276.2090812642587707, -215.2685392229145975 ) ) ;
#78521=CARTESIAN_POINT ( 'NONE',  ( -101.8775896937261365, -277.7536353275127112, -304.5255211627210770 ) ) ;
#78522=CARTESIAN_POINT ( 'NONE',  ( -67.01740533659108223, -291.8404474295331283, -199.3093585047412546 ) ) ;
#78523=CARTESIAN_POINT ( 'NONE',  ( -3.021931480836714368, -278.5818066254904579, -203.0304868062031858 ) ) ;
#78524=CARTESIAN_POINT ( 'NONE',  ( -81.92865648480223228, -291.2961625524351348, -207.5837070186526319 ) ) ;
#78525=CARTESIAN_POINT ( 'NONE',  ( -91.84026347515181499, -290.3089997870071102, -221.4208454254958269 ) ) ;
#78526=CARTESIAN_POINT ( 'NONE',  ( -19.78094129014038316, -292.8263582765110868, -343.3297327393677278 ) ) ;
#78529=CARTESIAN_POINT ( 'NONE',  ( -0.05415658918259873278, -292.0705723706474259, -207.5309696578219700 ) ) ;
#78531=CARTESIAN_POINT ( 'NONE',  ( -53.35057174420112602, -274.7666405000204009, -340.3538533559490702 ) ) ;
#78532=CARTESIAN_POINT ( 'NONE',  ( -114.0739551433859162, -295.6563977908514289, -266.7344052728408883 ) ) ;
#78533=CARTESIAN_POINT ( 'NONE',  ( -93.56876060867189437, -286.5789179362483878, -218.4007432970724949 ) ) ;
#78534=CARTESIAN_POINT ( 'NONE',  ( -7.014568142378860394, -286.2948331066494916, -203.9450938034151477 ) ) ;
#78535=CARTESIAN_POINT ( 'NONE',  ( 36.06705071093982440, -276.9804742235096455, -263.3355728474290345 ) ) ;
#78536=CARTESIAN_POINT ( 'NONE',  ( -91.62022021752939338, -293.8498222468210770, -321.6770628179526739 ) ) ;
#78537=CARTESIAN_POINT ( 'NONE',  ( -71.37710732562911176, -297.2680960404190387, -336.0986929038641051 ) ) ;
#78538=CARTESIAN_POINT ( 'NONE',  ( -35.12091352673736111, -275.8185683224580771, -343.7245871800645887 ) ) ;
#78541=CARTESIAN_POINT ( 'NONE',  ( -111.5727549941722856, -295.9634691978630485, -290.7448071737853184 ) ) ;
#78542=CARTESIAN_POINT ( 'NONE',  ( 31.27990846049819140, -289.0910839383534494, -241.3765798627018455 ) ) ;
#78544=CARTESIAN_POINT ( 'NONE',  ( 30.58297040466815275, -288.5662305582638396, -297.5186336925636965 ) ) ;
#78546=CARTESIAN_POINT ( 'NONE',  ( -95.71904859990847569, -278.2855413540873428, -220.4921068311262218 ) ) ;
#78547=CARTESIAN_POINT ( 'NONE',  ( -68.17768083229086074, -296.0980213357907473, -340.8058131758902505 ) ) ;
#78548=CARTESIAN_POINT ( 'NONE',  ( -56.99372731946348836, -287.4424358860316033, -343.5870827309071842 ) ) ;
#78550=CARTESIAN_POINT ( 'NONE',  ( -114.3168621293517475, -296.8948668174932664, -269.6069785302972264 ) ) ;
#78551=CARTESIAN_POINT ( 'NONE',  ( 27.50336777494408125, -293.4289877681877101, -236.7872493443745725 ) ) ;
#78555=CARTESIAN_POINT ( 'NONE',  ( -45.92834899839301244, -290.6791317570819615, -346.2357759003624551 ) ) ;
#78556=CARTESIAN_POINT ( 'NONE',  ( 25.22466315766300227, -278.6948066931273047, -320.2154176792147382 ) ) ;
#78557=CARTESIAN_POINT ( 'NONE',  ( -111.9849665934233087, -278.1329108403559758, -251.8221090231298547 ) ) ;
#78558=CARTESIAN_POINT ( 'NONE',  ( -74.69023864502166532, -285.5501706050789608, -335.2670175365548175 ) ) ;
#78559=CARTESIAN_POINT ( 'NONE',  ( 2.449775781553417353, -285.1492393251827480, -205.1288810338072324 ) ) ;
#78560=CARTESIAN_POINT ( 'NONE',  ( -53.74925661647637298, -287.3441958255147028, -342.9703893254933860 ) ) ;
#78561=CARTESIAN_POINT ( 'NONE',  ( 19.90280020763823643, -278.0943303123561918, -320.0131364649568582 ) ) ;
#78563=CARTESIAN_POINT ( 'NONE',  ( -110.1586453576392586, -278.6203065851875067, -265.1946407073208434 ) ) ;
#78564=CARTESIAN_POINT ( 'NONE',  ( -57.13285038070998922, -279.1385548112180004, -199.9892270064146373 ) ) ;
#78565=CARTESIAN_POINT ( 'NONE',  ( 26.66497348911988041, -276.0740402482012428, -228.1161390849143231 ) ) ;
#78566=CARTESIAN_POINT ( 'NONE',  ( -73.56426780823311162, -278.3773725683269049, -202.8485842138100850 ) ) ;
#78567=CARTESIAN_POINT ( 'NONE',  ( 183.2361720774044613, 262.7496117309314059, -151.9803302442668951 ) ) ;
#78568=CARTESIAN_POINT ( 'NONE',  ( -35.54135695043370902, -275.0154406052131435, -193.6044353622344261 ) ) ;
#78569=CARTESIAN_POINT ( 'NONE',  ( -75.50150854586291871, -298.9792230066044567, -204.1004214932385707 ) ) ;
#78570=CARTESIAN_POINT ( 'NONE',  ( 10.64812456238590066, -284.9090924074130271, -330.4860931364851808 ) ) ;
#78573=CARTESIAN_POINT ( 'NONE',  ( -44.06636157217130290, -287.0448043071465918, -197.3610837218801635 ) ) ;
#78574=CARTESIAN_POINT ( 'NONE',  ( -64.21013188906239577, -287.4665165483907003, -199.2692805856398479 ) ) ;
#78575=CARTESIAN_POINT ( 'NONE',  ( 3.664936194092168531, -287.8330935431459352, -330.9394921323816448 ) ) ;
#78576=CARTESIAN_POINT ( 'NONE',  ( -71.71687635028065699, -283.0018946269506728, -339.1933354625257948 ) ) ;
#78577=CARTESIAN_POINT ( 'NONE',  ( -30.16452048410592823, -278.5441904678078799, -196.8600337954603390 ) ) ;
#78578=CARTESIAN_POINT ( 'NONE',  ( -55.07396886762415278, -287.6822672812605788, -198.2216487374095095 ) ) ;
#78579=CARTESIAN_POINT ( 'NONE',  ( 36.21306841039208990, -279.9729961450294695, -265.8440640564992918 ) ) ;
#78580=CARTESIAN_POINT ( 'NONE',  ( -26.93524262507619937, -278.2322350932514041, -343.1137751119311474 ) ) ;
#78581=CARTESIAN_POINT ( 'NONE',  ( 34.76893079480420568, -276.2033946081338058, -282.4162377614863431 ) ) ;
#78582=CARTESIAN_POINT ( 'NONE',  ( 18.34556971237548595, -287.0691897059519988, -322.9627975774164383 ) ) ;
#78583=CARTESIAN_POINT ( 'NONE',  ( 24.13207741950450469, -282.9698058218727965, -316.4602882031379636 ) ) ;
#78584=CARTESIAN_POINT ( 'NONE',  ( -69.15528092880882127, -283.9518412852310121, -340.4285211352772649 ) ) ;
#78585=CARTESIAN_POINT ( 'NONE',  ( 0.3981328123779520611, -280.7364921607378960, -207.8149652685710578 ) ) ;
#78589=CARTESIAN_POINT ( 'NONE',  ( -7.386134101901441262, -290.5239463344674959, -339.9665793633228077 ) ) ;
#78590=CARTESIAN_POINT ( 'NONE',  ( -19.48551063167111508, -290.9618655087073193, -195.9127275134494255 ) ) ;
#78591=CARTESIAN_POINT ( 'NONE',  ( -38.07272056362097601, -273.1015159515761184, -197.1294714216506350 ) ) ;
#78592=CARTESIAN_POINT ( 'NONE',  ( 37.68264218367406215, -293.1127726809691012, -287.2924193020761550 ) ) ;
#78593=CARTESIAN_POINT ( 'NONE',  ( -109.9566051638406066, -289.1999716456214173, -257.5090153100776433 ) ) ;
#78594=CARTESIAN_POINT ( 'NONE',  ( 20.99526049813713513, -291.1585681003528521, -224.7909161590257554 ) ) ;
#78595=CARTESIAN_POINT ( 'NONE',  ( 22.29322579196597331, -289.3521155635723403, -313.1490381937547340 ) ) ;
#78596=CARTESIAN_POINT ( 'NONE',  ( 31.95455697924148097, -289.6233781216988064, -236.9535640164627637 ) ) ;
#78597=CARTESIAN_POINT ( 'NONE',  ( -67.23275674053692796, -291.4442404964923981, -339.1472022281287195 ) ) ;
#78598=CARTESIAN_POINT ( 'NONE',  ( -85.32271174349304488, -289.3912532321893423, -212.4329379963150757 ) ) ;
#78599=CARTESIAN_POINT ( 'NONE',  ( -3.929301603794604247, -294.4929273803697356, -203.2008337922928547 ) ) ;
#78600=CARTESIAN_POINT ( 'NONE',  ( -96.77276472027713794, -286.0901515181005266, -227.5453627034338524 ) ) ;
#78601=CARTESIAN_POINT ( 'NONE',  ( 5.431568940963765080, -294.6298804038204366, -208.5511197839680335 ) ) ;
#78604=CARTESIAN_POINT ( 'NONE',  ( 95.99055701654010875, -301.6291247887334634, -194.7578621600179929 ) ) ;
#78605=CARTESIAN_POINT ( 'NONE',  ( -43.11151744647708028, -281.1247050258659783, -345.1903128854513056 ) ) ;
#78606=CARTESIAN_POINT ( 'NONE',  ( -113.0465804601180935, -295.5807438471168211, -283.8122924865294294 ) ) ;
#78607=CARTESIAN_POINT ( 'NONE',  ( -3.623301486488966994, -272.7432604246999404, -204.4602919311154778 ) ) ;
#78608=CARTESIAN_POINT ( 'NONE',  ( -48.85420396401065091, -275.2796166150836825, -343.9579073213237166 ) ) ;
#78609=CARTESIAN_POINT ( 'NONE',  ( -65.77889535242896102, -298.9873643423164822, -202.5926193527098178 ) ) ;
#78610=CARTESIAN_POINT ( 'NONE',  ( -109.3595167034088291, -298.1761501539551205, -255.1740218110153364 ) ) ;
#78613=CARTESIAN_POINT ( 'NONE',  ( -97.30988669899636534, -296.7718875031885659, -312.2707627741876308 ) ) ;
#78616=CARTESIAN_POINT ( 'NONE',  ( 0.7132904829745017050, -284.5769898918645140, -205.3059286568074242 ) ) ;
#78617=CARTESIAN_POINT ( 'NONE',  ( -69.25753617374633109, -297.6201171569708208, -204.7076381851705378 ) ) ;
#78618=CARTESIAN_POINT ( 'NONE',  ( 23.86143494046273261, -286.9289598736797871, -223.6150281175455063 ) ) ;
#78620=CARTESIAN_POINT ( 'NONE',  ( 36.36392197253956482, -287.4982128966321966, -292.6155733824336380 ) ) ;
#78621=CARTESIAN_POINT ( 'NONE',  ( -112.1451423713069175, -298.6483663263388735, -261.2588198902338945 ) ) ;
#78622=CARTESIAN_POINT ( 'NONE',  ( -14.25725425521069312, -290.3520520566124787, -199.1772940938574834 ) ) ;
#78623=CARTESIAN_POINT ( 'NONE',  ( -99.29160707250838414, -278.3545621805811265, -224.8815966733992582 ) ) ;
#78624=CARTESIAN_POINT ( 'NONE',  ( 31.98288692825982693, -284.6237833571632905, -237.0123917617630980 ) ) ;
#78626=CARTESIAN_POINT ( 'NONE',  ( 34.67077106938914710, -286.5340918236167909, -284.6152590400130293 ) ) ;
#78628=CARTESIAN_POINT ( 'NONE',  ( -72.12226116782585450, -287.5119327589609384, -336.8234529237187758 ) ) ;
#78629=CARTESIAN_POINT ( 'NONE',  ( -106.0698082391928949, -274.4259209203800651, -243.6278728434055836 ) ) ;
#78630=CARTESIAN_POINT ( 'NONE',  ( 27.34280263180543713, -282.4395665715327937, -229.5861874555359350 ) ) ;
#78631=CARTESIAN_POINT ( 'NONE',  ( -85.36686949053191142, -293.7322676185532941, -328.4299556451662170 ) ) ;
#78632=CARTESIAN_POINT ( 'NONE',  ( 34.70355992560354252, -281.7073886536329610, -282.1288919350506603 ) ) ;
#78633=CARTESIAN_POINT ( 'NONE',  ( -111.5914549869816170, -296.4633496286864442, -290.7565563919953888 ) ) ;
#78634=CARTESIAN_POINT ( 'NONE',  ( -35.81677508070058025, -299.5917038824570113, -196.6673763113564348 ) ) ;
#78635=CARTESIAN_POINT ( 'NONE',  ( -33.77045976182287745, -284.1766139314307793, -194.8855560963399398 ) ) ;
#78637=CARTESIAN_POINT ( 'NONE',  ( -5.808665093568579962, -282.4668990852031811, -202.3121036303590472 ) ) ;
#78638=CARTESIAN_POINT ( 'NONE',  ( -104.9749334234064690, -295.9864081889618888, -242.2692294463513178 ) ) ;
#78639=VERTEX_POINT ( 'NONE', #34724 ) ;
#78641=CARTESIAN_POINT ( 'NONE',  ( 22.33984531576784605, -284.1478982837167564, -315.2148254123349034 ) ) ;
#78643=CARTESIAN_POINT ( 'NONE',  ( 10.64812456238590777, -284.1952119285918457, -210.2361428286349110 ) ) ;
#78644=CARTESIAN_POINT ( 'NONE',  ( 37.78966514558979384, -274.5466797099522864, -254.1918373951729393 ) ) ;
#78645=CARTESIAN_POINT ( 'NONE',  ( 20.18420522177757093, -292.7517713517248694, -225.3990266266529829 ) ) ;
#78646=CARTESIAN_POINT ( 'NONE',  ( 17.56660933272043934, -282.3756588339055611, -221.2104790707151665 ) ) ;
#78647=CARTESIAN_POINT ( 'NONE',  ( 36.15253068161145933, -277.2398576587238495, -277.0721873236410602 ) ) ;
#78648=CARTESIAN_POINT ( 'NONE',  ( -47.16251540386964791, -284.5998663077435822, -346.1381453669321786 ) ) ;
#78649=CARTESIAN_POINT ( 'NONE',  ( 31.44779713559346135, -280.0058057405393015, -244.6196081082668172 ) ) ;
#78650=CARTESIAN_POINT ( 'NONE',  ( -90.48549324443042963, -279.8044037137273676, -323.3568377834724856 ) ) ;
#78651=CARTESIAN_POINT ( 'NONE',  ( -3.410510378925430963, -298.4659870783543738, -193.3611102151625971 ) ) ;
#78652=CARTESIAN_POINT ( 'NONE',  ( 37.94583847598392623, -275.1827293055648624, -254.1498913486779827 ) ) ;
#78653=CARTESIAN_POINT ( 'NONE',  ( 9.146153794915321100, -296.3287442250542654, -328.5668153844217159 ) ) ;
#78656=CARTESIAN_POINT ( 'NONE',  ( -112.7168167278714606, -294.5941923707146657, -278.0355740972362355 ) ) ;
#78657=CARTESIAN_POINT ( 'NONE',  ( -48.87897666851846168, -273.4090085141683630, -198.1650496772829513 ) ) ;
#78658=CARTESIAN_POINT ( 'NONE',  ( 24.33738336087547438, -295.6741859404183970, -315.3097242076204338 ) ) ;
#78659=CARTESIAN_POINT ( 'NONE',  ( -5.946334098559480807, -295.8536164491032423, -340.2348591996635037 ) ) ;
#78660=CARTESIAN_POINT ( 'NONE',  ( -10.03188028773695706, -290.6950696752558656, -340.0888085637946006 ) ) ;
#78661=CARTESIAN_POINT ( 'NONE',  ( -109.9571255299280779, -276.3185844365544312, -288.4979446519641328 ) ) ;
#78662=CARTESIAN_POINT ( 'NONE',  ( 16.65900263320595442, -278.1965477615525515, -321.5981973212766434 ) ) ;
#78663=CARTESIAN_POINT ( 'NONE',  ( -85.42656270510117622, -293.8022973010352530, -327.2545164187904447 ) ) ;
#78664=CARTESIAN_POINT ( 'NONE',  ( 28.20590577343461547, -282.9103457800706565, -232.3635280711608004 ) ) ;
#78665=CARTESIAN_POINT ( 'NONE',  ( -94.35379629054345685, -284.1217069907488053, -224.2560132696502819 ) ) ;
#78666=CARTESIAN_POINT ( 'NONE',  ( 195.6954042328585501, 277.0390073305854912, -125.2964528022664723 ) ) ;
#78668=CARTESIAN_POINT ( 'NONE',  ( -72.38043005085809511, -285.2416333511620223, -206.2815022803524698 ) ) ;
#78669=CARTESIAN_POINT ( 'NONE',  ( 37.67940328304122488, -282.4311732373903396, -254.3821097311873700 ) ) ;
#78670=CARTESIAN_POINT ( 'NONE',  ( -68.32601142235476743, -284.4490657676504384, -200.2898321480615778 ) ) ;
#78671=CARTESIAN_POINT ( 'NONE',  ( -110.3297187660448344, -279.7954009736042735, -246.4106218731513138 ) ) ;
#78672=CARTESIAN_POINT ( 'NONE',  ( -64.82710012619783413, -278.9246673186498242, -341.6015836978963875 ) ) ;
#78674=CARTESIAN_POINT ( 'NONE',  ( 27.33386217378598815, -273.4809262143061233, -301.5434626090942629 ) ) ;
#78675=CARTESIAN_POINT ( 'NONE',  ( -103.3473159737818605, -256.7681506039956503, -326.7728887287452153 ) ) ;
#78677=CARTESIAN_POINT ( 'NONE',  ( -108.0467196094137705, -274.8703032242514155, -245.8493117315155985 ) ) ;
#78679=CARTESIAN_POINT ( 'NONE',  ( -54.85476745283906297, -277.8461547975692838, -197.7464701284746695 ) ) ;
#78680=CARTESIAN_POINT ( 'NONE',  ( -66.64564125943893202, -293.4336512280216880, -200.2522522877451081 ) ) ;
#78681=CARTESIAN_POINT ( 'NONE',  ( 18.55988834123604647, -292.2324456558302472, -223.2558627014914805 ) ) ;
#78682=CARTESIAN_POINT ( 'NONE',  ( -102.2527158509085865, -289.5168496268728404, -311.7639759952966187 ) ) ;
#78684=CARTESIAN_POINT ( 'NONE',  ( -27.83924711164970489, -293.5086117438322049, -346.2316098671840905 ) ) ;
#78685=CARTESIAN_POINT ( 'NONE',  ( -71.53093684184175061, -283.9924688108109194, -204.9582395309947742 ) ) ;
#78686=CARTESIAN_POINT ( 'NONE',  ( -5.533500342538035355, -294.3354709628830506, -203.2717455720560054 ) ) ;
#78687=CARTESIAN_POINT ( 'NONE',  ( -0.9936351311795564856, -283.8739487287514294, -334.2364782509478687 ) ) ;
#78689=CARTESIAN_POINT ( 'NONE',  ( -92.65090200224467765, -292.2250305152729197, -217.0528558285718077 ) ) ;
#78690=CARTESIAN_POINT ( 'NONE',  ( -19.52561274059026886, -280.7797560442970735, -199.4527658493097704 ) ) ;
#78691=CARTESIAN_POINT ( 'NONE',  ( 37.96406132851063120, -292.5244393928860518, -284.4694049368013680 ) ) ;
#78692=CARTESIAN_POINT ( 'NONE',  ( 35.79719336610538960, -288.6518225984476658, -293.9166073397963146 ) ) ;
#78693=CARTESIAN_POINT ( 'NONE',  ( -36.08155718505700804, -289.5291274786713416, -347.3023591951497338 ) ) ;
#78694=CARTESIAN_POINT ( 'NONE',  ( 32.66936623805344908, -287.4447295021695936, -249.6421478981004327 ) ) ;
#78697=CARTESIAN_POINT ( 'NONE',  ( 18.63338050518334299, -296.1187078977703209, -321.4972915332950834 ) ) ;
#78698=CARTESIAN_POINT ( 'NONE',  ( -80.33397150388192642, -296.1681898797301642, -207.0126538561590621 ) ) ;
#78699=CARTESIAN_POINT ( 'NONE',  ( -108.4032997511616827, -277.3773216427051125, -288.1232286798413611 ) ) ;
#78700=CARTESIAN_POINT ( 'NONE',  ( -110.0416630628048722, -272.3775680725170787, -245.1769504869315597 ) ) ;
#78701=CARTESIAN_POINT ( 'NONE',  ( -55.99734827041613983, -293.7765201471142404, -341.7068815860121163 ) ) ;
#78702=CARTESIAN_POINT ( 'NONE',  ( 23.09551691191135347, -276.7238227006940861, -227.6154611429739134 ) ) ;
#78703=CARTESIAN_POINT ( 'NONE',  ( -104.3093292422995120, -271.1177815792476054, -238.3267282077571849 ) ) ;
#78704=CARTESIAN_POINT ( 'NONE',  ( 35.60333806118509870, -294.8698147224025092, -278.9418042655849490 ) ) ;
#78705=CARTESIAN_POINT ( 'NONE',  ( -61.10040065245200225, -296.4475079153704087, -339.7672783022074441 ) ) ;
#78707=CARTESIAN_POINT ( 'NONE',  ( -92.36522679112401590, -293.8367803855977058, -321.5898463016061442 ) ) ;
#78708=CARTESIAN_POINT ( 'NONE',  ( -114.0206494304582776, -273.4265779991619070, -264.6484528472711872 ) ) ;
#78709=CARTESIAN_POINT ( 'NONE',  ( 8.331570025339173569, -286.9875060328600398, -328.0614412823993007 ) ) ;
#78711=CARTESIAN_POINT ( 'NONE',  ( -78.81366317373289121, -274.0015311204903128, -205.5567725705720079 ) ) ;
#78712=CARTESIAN_POINT ( 'NONE',  ( -109.0672412583592461, -297.0669115010791757, -256.6001894047518590 ) ) ;
#78713=CARTESIAN_POINT ( 'NONE',  ( -9.492924349842045473, -282.3941804789812977, -200.3407460104639881 ) ) ;
#78714=CARTESIAN_POINT ( 'NONE',  ( 22.50013162796342669, -279.5944832560663826, -222.6721243455703814 ) ) ;
#78716=CARTESIAN_POINT ( 'NONE',  ( -52.90510366941208531, -282.5950364036022506, -345.7222005599020349 ) ) ;
#78717=CARTESIAN_POINT ( 'NONE',  ( 35.10214353962329170, -275.2284586123627719, -296.3095383389904214 ) ) ;
#78718=CARTESIAN_POINT ( 'NONE',  ( -7.827833069119636278, -278.8323497611644370, -200.0947582849837829 ) ) ;
#78719=CARTESIAN_POINT ( 'NONE',  ( -3.199561070060736867, -278.5018131531216454, -203.3815033874062692 ) ) ;
#78721=CARTESIAN_POINT ( 'NONE',  ( -6.263764471634402753, -273.0434147924614194, -203.6562693263288963 ) ) ;
#78722=CARTESIAN_POINT ( 'NONE',  ( 36.27544832617159898, -277.3673985747126380, -255.9597078771451208 ) ) ;
#78724=CARTESIAN_POINT ( 'NONE',  ( -4.025340937891983550, -290.5093937367022363, -202.7567480277062657 ) ) ;
#78725=CARTESIAN_POINT ( 'NONE',  ( -96.57886909800195951, -291.2138277587417861, -221.1476754266053604 ) ) ;
#78726=CARTESIAN_POINT ( 'NONE',  ( -31.56512130915528047, -278.9796750362481248, -345.3568645040633669 ) ) ;
#78727=CARTESIAN_POINT ( 'NONE',  ( -5.661632698341396264, -272.4686196240838854, -202.3804296913274072 ) ) ;
#78729=( LENGTH_UNIT ( ) NAMED_UNIT ( * ) SI_UNIT ( .MILLI., .METRE. ) );
#78730=CARTESIAN_POINT ( 'NONE',  ( -33.23510068027243136, -284.1035756449785481, -195.4232692572382746 ) ) ;
#78732=CARTESIAN_POINT ( 'NONE',  ( -42.43250118660234449, -293.9127061532680045, -343.5814310777573155 ) ) ;
#78733=CARTESIAN_POINT ( 'NONE',  ( 32.55457183249233566, -286.0191731522660348, -295.3686497511686184 ) ) ;
#78736=CARTESIAN_POINT ( 'NONE',  ( 7.231656944940937137, -292.4450679508937014, -330.7434545395724399 ) ) ;
#78737=CARTESIAN_POINT ( 'NONE',  ( -110.8290274778271822, -282.7721886963385032, -290.9115552692520055 ) ) ;
#78738=CARTESIAN_POINT ( 'NONE',  ( -91.90184341310330751, -280.8571202821070756, -220.6657340871182384 ) ) ;
#78739=CARTESIAN_POINT ( 'NONE',  ( -80.72602444033948643, -286.6833048952634613, -207.1638184653175472 ) ) ;
#78740=CARTESIAN_POINT ( 'NONE',  ( 34.96037288133486953, -287.6861962870319189, -280.5223947339177357 ) ) ;
#78741=CARTESIAN_POINT ( 'NONE',  ( -35.08149971586499305, -278.4484910029231628, -343.9156311861027007 ) ) ;
#78742=CARTESIAN_POINT ( 'NONE',  ( -93.22013547409262912, -280.0248114800314170, -223.1168271366433942 ) ) ;
#78744=CARTESIAN_POINT ( 'NONE',  ( 4.250369349333530167, -288.5892934095487590, -207.4618369971614413 ) ) ;
#78745=AXIS2_PLACEMENT_3D ( 'NONE', #77362, #28125, #62721 ) ;
#78747=CARTESIAN_POINT ( 'NONE',  ( -102.3152563265819168, -296.9270779397500064, -229.0399732813357332 ) ) ;
#78749=CARTESIAN_POINT ( 'NONE',  ( 29.71619581586000791, -289.9663765324426663, -303.1496127807340599 ) ) ;
#78751=CARTESIAN_POINT ( 'NONE',  ( 25.18497378105907814, -283.4090924074130839, -220.4570493818173702 ) ) ;
#78753=CARTESIAN_POINT ( 'NONE',  ( -24.44841109318233308, -272.2160532570519536, -196.2556116564043123 ) ) ;
#78754=CARTESIAN_POINT ( 'NONE',  ( 21.60350459938456780, -291.2967998708135156, -222.0713337848848994 ) ) ;
#78755=CARTESIAN_POINT ( 'NONE',  ( -86.53603409076498565, -295.2656914877719032, -324.3787627616300142 ) ) ;
#78756=CARTESIAN_POINT ( 'NONE',  ( 18.28696722790054352, -288.3896727451667630, -222.0272879884981592 ) ) ;
#78757=CARTESIAN_POINT ( 'NONE',  ( 34.93475296403097730, -283.5196923001047935, -286.3012668201505448 ) ) ;
#78758=CARTESIAN_POINT ( 'NONE',  ( -69.09575587127618235, -290.8869152356656969, -339.8756900397437448 ) ) ;
#78759=CARTESIAN_POINT ( 'NONE',  ( -112.8705217766124775, -291.7138354235013935, -282.5551892247387968 ) ) ;
#78760=CARTESIAN_POINT ( 'NONE',  ( -112.3170219535684424, -286.5087614312796518, -273.7533198087757569 ) ) ;
#78761=CARTESIAN_POINT ( 'NONE',  ( -110.6660150258689583, -278.4213414652741108, -294.0390468988787802 ) ) ;
#78762=CARTESIAN_POINT ( 'NONE',  ( -8.952198915101265086, -292.7637122573524380, -340.4404616936378716 ) ) ;
#78763=CARTESIAN_POINT ( 'NONE',  ( -8.859138326056228863, -280.2479547456487126, -198.8227109713326115 ) ) ;
#78764=CARTESIAN_POINT ( 'NONE',  ( -103.1360020772057027, -274.8739466727927834, -235.8698452527687266 ) ) ;
#78765=EDGE_CURVE ( 'NONE', #64529, #50851, #88127, .T. ) ;
#78766=CARTESIAN_POINT ( 'NONE',  ( -20.19161114001083490, -291.3376638359845856, -345.3538533559490702 ) ) ;
#78767=CARTESIAN_POINT ( 'NONE',  ( 25.32177333006835340, -273.2169968841843684, -227.3582471649257570 ) ) ;
#78769=CARTESIAN_POINT ( 'NONE',  ( 33.38149988018159320, -281.3022602403335100, -288.7471666906474752 ) ) ;
#78770=CARTESIAN_POINT ( 'NONE',  ( 35.34827300217931878, -276.4494912237666995, -246.0242691206248082 ) ) ;
#78771=CARTESIAN_POINT ( 'NONE',  ( -101.7388919048687796, -298.4602637870092394, -234.7468426564614106 ) ) ;
#78772=CARTESIAN_POINT ( 'NONE',  ( -79.04199218841267793, -282.6586478207116784, -334.8119197978743955 ) ) ;
#78773=CARTESIAN_POINT ( 'NONE',  ( -104.4848757726212085, -292.7268833308195894, -239.2200201331006610 ) ) ;
#78774=CARTESIAN_POINT ( 'NONE',  ( -36.96437105546868906, -275.6569558883413151, -194.1491333638721812 ) ) ;
#78775=CARTESIAN_POINT ( 'NONE',  ( -89.83674463381768760, -274.6452151841528462, -214.6329514324554282 ) ) ;
#78777=CARTESIAN_POINT ( 'NONE',  ( 17.52010263984465865, -296.2658354158406837, -321.2552337926327937 ) ) ;
#78778=CARTESIAN_POINT ( 'NONE',  ( -109.5364183966800908, -282.2975897107580749, -290.1060335739248330 ) ) ;
#78779=CARTESIAN_POINT ( 'NONE',  ( -114.2303868047341808, -290.1722751346385962, -274.0859203373668720 ) ) ;
#78780=CARTESIAN_POINT ( 'NONE',  ( 37.28787442950225284, -273.5528023500567656, -268.8533378336859982 ) ) ;
#78781=CARTESIAN_POINT ( 'NONE',  ( 35.91639016150526942, -288.8845141295504959, -249.2050913817516005 ) ) ;
#78782=CARTESIAN_POINT ( 'NONE',  ( -101.3870638784975711, -289.9594237387763656, -234.5859267401124271 ) ) ;
#78784=CARTESIAN_POINT ( 'NONE',  ( -101.8139284062927601, -288.5840749097957882, -311.4699592090917122 ) ) ;
#78785=CARTESIAN_POINT ( 'NONE',  ( -107.7473328911050459, -289.9608120914307960, -289.9158785394840265 ) ) ;
#78787=CARTESIAN_POINT ( 'NONE',  ( 32.58867012579311506, -289.0355857338158785, -301.8450158519042930 ) ) ;
#78788=CARTESIAN_POINT ( 'NONE',  ( 18.32728339696601694, -276.5571478352205190, -317.6162950548729214 ) ) ;
#78789=CARTESIAN_POINT ( 'NONE',  ( 21.12304930792435798, -293.1442356326679715, -319.9934218183161647 ) ) ;
#78790=CARTESIAN_POINT ( 'NONE',  ( -102.5028351540022271, -285.4222619314238045, -229.3761112896763734 ) ) ;
#78791=CARTESIAN_POINT ( 'NONE',  ( 34.25225138021647098, -282.0757264132767546, -284.7904662526069046 ) ) ;
#78792=CARTESIAN_POINT ( 'NONE',  ( 64.77658176787873856, 47.97751566260769351, -318.9316874262945589 ) ) ;
#78793=CARTESIAN_POINT ( 'NONE',  ( -23.26540662898876732, -107.7375312792409972, -361.8887297295785288 ) ) ;
#78794=CARTESIAN_POINT ( 'NONE',  ( -106.1534499783927572, -259.7701228362822690, -315.4954753543551078 ) ) ;
#78795=CARTESIAN_POINT ( 'NONE',  ( -34.02314740851217323, -273.2921226783739712, -197.2749432629602779 ) ) ;
#78796=CARTESIAN_POINT ( 'NONE',  ( -46.20256731205039102, -272.8574258610898369, -197.5894812963507832 ) ) ;
#78797=CARTESIAN_POINT ( 'NONE',  ( -95.53906058955573144, -295.3794392362768235, -320.6860038612025505 ) ) ;
#78798=CARTESIAN_POINT ( 'NONE',  ( -75.91738900125099576, -208.6651993415634081, -353.8496858908021068 ) ) ;
#78799=CARTESIAN_POINT ( 'NONE',  ( 0.9631155154215390590, -273.2369321440110639, -204.1187490609767963 ) ) ;
#78800=CARTESIAN_POINT ( 'NONE',  ( -73.46837056570362279, -299.4278360822341938, -205.5095245980904792 ) ) ;
#78801=CARTESIAN_POINT ( 'NONE',  ( 10.44856727470821234, -289.6915794273643314, -326.2615094317041553 ) ) ;
#78802=CARTESIAN_POINT ( 'NONE',  ( -110.6773800185677032, -291.6567055389387519, -268.4674349851497368 ) ) ;
#78804=CARTESIAN_POINT ( 'NONE',  ( -104.3915305150653410, -297.0060870749479705, -307.8480964781485341 ) ) ;
#78805=CARTESIAN_POINT ( 'NONE',  ( -35.93856748887137798, -286.5625707395337827, -197.3130539380764503 ) ) ;
#78806=CARTESIAN_POINT ( 'NONE',  ( 8.817326177506853213, -295.2398443936248782, -331.7899638982167403 ) ) ;
#78807=CARTESIAN_POINT ( 'NONE',  ( -44.78342606498735989, -295.6361621060548828, -346.9922044147858173 ) ) ;
#78808=CARTESIAN_POINT ( 'NONE',  ( 27.48556370688076456, -293.2624134424286808, -236.7988494633435153 ) ) ;
#78810=CARTESIAN_POINT ( 'NONE',  ( -95.83714058952023152, -275.1268382058628390, -222.5120833378332179 ) ) ;
#78813=CARTESIAN_POINT ( 'NONE',  ( -107.3605141159134604, -278.4691808941695399, -238.3441166582337019 ) ) ;
#78814=CARTESIAN_POINT ( 'NONE',  ( 34.35897646600415811, -274.1807475357840644, -287.8915151973031925 ) ) ;
#78815=CARTESIAN_POINT ( 'NONE',  ( 30.50050871200883051, -276.8633059683416491, -298.0794949333244404 ) ) ;
#78816=CARTESIAN_POINT ( 'NONE',  ( -34.16824712897884808, -275.8516850649032790, -194.4407438300254682 ) ) ;
#78818=CARTESIAN_POINT ( 'NONE',  ( 36.34250494505783280, -273.3698105997611947, -254.5188725013404678 ) ) ;
#78819=CARTESIAN_POINT ( 'NONE',  ( -108.2758702109818785, -297.4370336704475335, -252.6396406791724303 ) ) ;
#78820=CARTESIAN_POINT ( 'NONE',  ( -97.67680051326463797, -294.5441423895704816, -312.4924671092201152 ) ) ;
#78822=CARTESIAN_POINT ( 'NONE',  ( -99.59627549111229428, -278.4439350502482853, -315.5929721016261169 ) ) ;
#78823=CARTESIAN_POINT ( 'NONE',  ( -5.064173771200484175, -276.7817252548840088, -335.8514264305433699 ) ) ;
#78824=CARTESIAN_POINT ( 'NONE',  ( 35.38551671859860903, -285.9343379331483561, -246.4418350914553457 ) ) ;
#78825=CARTESIAN_POINT ( 'NONE',  ( -34.86135989402453816, -300.0832881303522868, -195.1935993454034133 ) ) ;
#78826=CARTESIAN_POINT ( 'NONE',  ( 82.64002947064351190, -300.2510188964802182, -197.7678940087098454 ) ) ;
#78827=CARTESIAN_POINT ( 'NONE',  ( 5.931921739323415821, -287.6457775068022329, -329.4157334304510982 ) ) ;
#78828=CARTESIAN_POINT ( 'NONE',  ( -6.324579191209457107, -278.7051285722065472, -203.1467440808307572 ) ) ;
#78829=CARTESIAN_POINT ( 'NONE',  ( -24.75793025553718962, -278.7905718417633807, -197.8557826513423379 ) ) ;
#78830=CARTESIAN_POINT ( 'NONE',  ( -3.264513540184294182, -284.6023387384749981, -337.1865673937621750 ) ) ;
#78831=CARTESIAN_POINT ( 'NONE',  ( -71.82724894726753462, -278.7237059831081183, -335.1663219729223897 ) ) ;
#78833=CARTESIAN_POINT ( 'NONE',  ( 35.29383523686740887, -274.2445745864573041, -293.3941251146179070 ) ) ;
#78834=CARTESIAN_POINT ( 'NONE',  ( 29.17535785020994510, -275.7938614549270255, -239.9175198899723966 ) ) ;
#78835=CARTESIAN_POINT ( 'NONE',  ( 23.10197250560197091, -282.9439607906085712, -225.6778899466615940 ) ) ;
#78837=CARTESIAN_POINT ( 'NONE',  ( 37.54479479385048535, -289.3440152264710719, -260.2949828763424875 ) ) ;
#78838=CARTESIAN_POINT ( 'NONE',  ( 4.793351120182042457, -292.4833538933152681, -332.4682561183909115 ) ) ;
#78840=CARTESIAN_POINT ( 'NONE',  ( -29.92354717195936331, -272.8328310150862990, -197.2433056211007738 ) ) ;
#78841=CARTESIAN_POINT ( 'NONE',  ( -22.47041274133773570, -290.3841489371648663, -197.6307234492704765 ) ) ;
#78842=CARTESIAN_POINT ( 'NONE',  ( -49.37856652629597676, -155.6656457446864010, -366.7448178265262868 ) ) ;
#78844=CARTESIAN_POINT ( 'NONE',  ( -54.36593831843376279, -287.7467392801374899, -344.7986921315372797 ) ) ;
#78845=CARTESIAN_POINT ( 'NONE',  ( -3.914639667600360529, -284.7268310658551513, -202.1074524777421857 ) ) ;
#78846=CARTESIAN_POINT ( 'NONE',  ( -34.80821971631973355, -284.4450152945685204, -343.9192623047369466 ) ) ;
#78847=CARTESIAN_POINT ( 'NONE',  ( -89.00108409341792992, -284.6037231211263361, -322.2386801374091760 ) ) ;
#78848=CARTESIAN_POINT ( 'NONE',  ( -68.95659831317985322, -293.6184361392986943, -201.9445591541790748 ) ) ;
#78849=CARTESIAN_POINT ( 'NONE',  ( -32.68812320711818842, -274.4425430918141160, -193.5099041309908898 ) ) ;
#78850=CARTESIAN_POINT ( 'NONE',  ( -109.8434314805830496, -288.9039998675888228, -249.0817112723595415 ) ) ;
#78851=CARTESIAN_POINT ( 'NONE',  ( -71.57085032350299514, -277.4918688796414017, -339.3347743804868628 ) ) ;
#78852=CARTESIAN_POINT ( 'NONE',  ( -2.350907528260103074, -296.5666174542132012, -336.2966261577164460 ) ) ;
#78855=CARTESIAN_POINT ( 'NONE',  ( -106.0198643532816760, -283.5839705646019979, -244.1971497086835541 ) ) ;
#78856=CARTESIAN_POINT ( 'NONE',  ( -66.55920959481436228, -277.6693198048137106, -201.2862470725625883 ) ) ;
#78857=CARTESIAN_POINT ( 'NONE',  ( -113.6483667957982249, -271.0322748495758560, -270.3418062714382586 ) ) ;
#78858=CARTESIAN_POINT ( 'NONE',  ( -43.22354951157114300, -276.4769711681833542, -343.2260376357445466 ) ) ;
#78859=CARTESIAN_POINT ( 'NONE',  ( -5.761906345179846234, -293.9952320767264951, -203.7632424565805991 ) ) ;
#78860=CARTESIAN_POINT ( 'NONE',  ( 25.04203643358045284, -293.9651293498113773, -231.9024160321915247 ) ) ;
#78862=CARTESIAN_POINT ( 'NONE',  ( -58.69750209010320674, -296.6377533089294047, -343.8821592511580434 ) ) ;
#78863=CARTESIAN_POINT ( 'NONE',  ( -106.8699237221404132, -296.0885254884846631, -292.7694633599614917 ) ) ;
#78864=CARTESIAN_POINT ( 'NONE',  ( -7.397180472973788667, -290.6598054528595867, -339.1794754100254750 ) ) ;
#78865=CARTESIAN_POINT ( 'NONE',  ( -97.17105238061110128, -284.0685135171043498, -318.8529486178920251 ) ) ;
#78866=CARTESIAN_POINT ( 'NONE',  ( -91.27292320571639550, -271.4346562141673189, -217.1471286850362219 ) ) ;
#78867=CARTESIAN_POINT ( 'NONE',  ( -40.81434760645371540, -285.8430587348753988, -193.3872716976526078 ) ) ;
#78868=CARTESIAN_POINT ( 'NONE',  ( -48.83680483807923167, -279.1790349570469516, -344.1680478054839796 ) ) ;
#78870=CARTESIAN_POINT ( 'NONE',  ( -33.21344459669982996, -285.1640135841489609, -197.1922896316770561 ) ) ;
#78871=CARTESIAN_POINT ( 'NONE',  ( -72.26575763000421659, -287.5139771011550920, -336.7480090562880832 ) ) ;
#78872=CARTESIAN_POINT ( 'NONE',  ( 10.80643407470098794, -61.58976173765800155, -353.1561788127373802 ) ) ;
#78873=CARTESIAN_POINT ( 'NONE',  ( 30.02093982759445367, -286.6789709701212132, -241.9411504204626056 ) ) ;
#78875=CARTESIAN_POINT ( 'NONE',  ( -13.48365126673568959, -283.6910015016651982, -343.3242163065697241 ) ) ;
#78876=CARTESIAN_POINT ( 'NONE',  ( -107.0417464003678418, -290.0250958174759717, -238.0673917571192533 ) ) ;
#78877=CARTESIAN_POINT ( 'NONE',  ( -81.78891360139557776, -281.0579529140076147, -208.4669694056055960 ) ) ;
#78878=CARTESIAN_POINT ( 'NONE',  ( -112.7532461084423971, -280.0296876695396122, -257.4616216287933526 ) ) ;
#78879=CARTESIAN_POINT ( 'NONE',  ( -3.147213100939972197, -280.3504110376719609, -205.8509164363069885 ) ) ;
#78880=CARTESIAN_POINT ( 'NONE',  ( -31.22960994268312618, -276.1096044057277936, -195.9540361349819193 ) ) ;
#78881=CARTESIAN_POINT ( 'NONE',  ( 0.5405028384220336157, -294.5617322281331667, -337.4131433633274355 ) ) ;
#78882=CARTESIAN_POINT ( 'NONE',  ( -76.75821235114470653, -287.6028049805501041, -333.7502760934303865 ) ) ;
#78884=CARTESIAN_POINT ( 'NONE',  ( -71.82861590845720912, -293.2041853916803120, -202.3974742059271250 ) ) ;
#78885=CARTESIAN_POINT ( 'NONE',  ( -109.4486622139711613, -295.2978827748174808, -283.6523805615703964 ) ) ;
#78887=CARTESIAN_POINT ( 'NONE',  ( -1.718459570622664856, -284.4964707525649601, -335.7385166820840254 ) ) ;
#78888=CARTESIAN_POINT ( 'NONE',  ( -109.8260110367138225, -296.0969714280259382, -279.6043115475146692 ) ) ;
#78889=CARTESIAN_POINT ( 'NONE',  ( -27.90083520284281349, -293.2488765034984795, -194.2000875221678768 ) ) ;
#78890=CARTESIAN_POINT ( 'NONE',  ( 9.335259180758857411, -281.3645403619297554, -214.0354353454985414 ) ) ;
#78891=CARTESIAN_POINT ( 'NONE',  ( -64.80467480614187537, -272.7608827618702776, -198.6629112136309061 ) ) ;
#78892=CARTESIAN_POINT ( 'NONE',  ( -106.4182938034128796, -290.7677145646187000, -304.2717275767953424 ) ) ;
#78893=CARTESIAN_POINT ( 'NONE',  ( 0.2348261872157848540, -280.6969583256506553, -336.1659974276649905 ) ) ;
#78894=CARTESIAN_POINT ( 'NONE',  ( -95.64767900399191092, -291.5644882152136574, -220.0800782025988553 ) ) ;
#78895=CARTESIAN_POINT ( 'NONE',  ( -8.206155462136184298, -288.9931955268025945, -337.3719334296230841 ) ) ;
#78898=CARTESIAN_POINT ( 'NONE',  ( 173.5779064319110603, 240.4672869823826886, -177.0707307568671069 ) ) ;
#78899=CARTESIAN_POINT ( 'NONE',  ( -4.771743288812454686, -277.9809262143061233, -202.8022627189028810 ) ) ;
#78900=CARTESIAN_POINT ( 'NONE',  ( -110.4418981769703407, -277.7099087781375033, -273.3549068340353188 ) ) ;
#78902=CARTESIAN_POINT ( 'NONE',  ( -93.31736081847009245, -278.1426119315385677, -223.0031239198665958 ) ) ;
#78903=CARTESIAN_POINT ( 'NONE',  ( -24.15905243364050037, -273.8826642618506071, -194.4652750547240032 ) ) ;
#78904=CARTESIAN_POINT ( 'NONE',  ( -37.52155448479069122, -140.8893142108368295, -362.3101970415223150 ) ) ;
#78905=CARTESIAN_POINT ( 'NONE',  ( -98.94200552241284186, -277.7322230586455021, -225.1283281292398044 ) ) ;
#78906=CARTESIAN_POINT ( 'NONE',  ( -26.52888351673109213, -280.9341468423341439, -344.2710678366819934 ) ) ;
#78907=CARTESIAN_POINT ( 'NONE',  ( -112.6012921497164712, -298.4463838982779862, -259.7802429206159331 ) ) ;
#78908=CARTESIAN_POINT ( 'NONE',  ( 32.40741619691913655, -294.3324734275357741, -292.1108125454542801 ) ) ;
#78910=CARTESIAN_POINT ( 'NONE',  ( -70.20794647113758913, -288.1794116207494199, -336.1097920166418476 ) ) ;
#78911=CARTESIAN_POINT ( 'NONE',  ( 32.45704842535066348, -275.7887021480069052, -237.9628780341154766 ) ) ;
#78912=CARTESIAN_POINT ( 'NONE',  ( -63.08145301655268611, -297.8741905686242148, -201.9961077622904497 ) ) ;
#78913=VERTEX_POINT ( 'NONE', #13891 ) ;
#78917=CARTESIAN_POINT ( 'NONE',  ( -72.28912095828310669, -280.6578545327106440, -205.9180900315417375 ) ) ;
#78918=CARTESIAN_POINT ( 'NONE',  ( -1.631734303739330150, -282.2789878187024328, -203.2882295976607736 ) ) ;
#78919=CARTESIAN_POINT ( 'NONE',  ( -69.12208016560440171, -282.5394972001288352, -336.3553872796270525 ) ) ;
#78920=CARTESIAN_POINT ( 'NONE',  ( -49.36490895107633747, -281.7576888984771131, -197.1060299160584748 ) ) ;
#78921=CARTESIAN_POINT ( 'NONE',  ( -9.746533694308324058, -275.1649145764586706, -338.7064619056924926 ) ) ;
#78926=CARTESIAN_POINT ( 'NONE',  ( -106.1961321355999104, -278.9143613314565755, -304.5868961496231009 ) ) ;
#78930=CARTESIAN_POINT ( 'NONE',  ( -111.8647353856507607, -286.6791702598127358, -258.8482816898892906 ) ) ;
#78931=CARTESIAN_POINT ( 'NONE',  ( 27.29595319998228220, -293.2164570076552650, -304.7414272618611903 ) ) ;
#78932=CARTESIAN_POINT ( 'NONE',  ( 14.52882399755339549, -287.6938420228087239, -327.2026394220102929 ) ) ;
#78933=CARTESIAN_POINT ( 'NONE',  ( -103.1290018275198292, -283.2467187788606111, -236.4493951409342003 ) ) ;
#78934=CARTESIAN_POINT ( 'NONE',  ( -109.5612260839293270, -282.9419441419296390, -284.4931733608713103 ) ) ;
#78935=CARTESIAN_POINT ( 'NONE',  ( -78.75979019367456146, -287.8580833506096610, -331.7621786844200642 ) ) ;
#78936=CARTESIAN_POINT ( 'NONE',  ( 31.73347737416975889, -283.0876891809436984, -295.3257960551916881 ) ) ;
#78937=CARTESIAN_POINT ( 'NONE',  ( 26.80552617765052403, -273.0300826955864864, -231.4013386424830117 ) ) ;
#78939=CARTESIAN_POINT ( 'NONE',  ( -112.6931817981279238, -283.0997274476171128, -258.6738327191150120 ) ) ;
#78940=CARTESIAN_POINT ( 'NONE',  ( -101.3939463261774421, -298.0292207629465224, -309.3779144189761041 ) ) ;
#78941=CARTESIAN_POINT ( 'NONE',  ( -43.49028171077085858, -283.9746241944650365, -195.3943532962559289 ) ) ;
#78943=CARTESIAN_POINT ( 'NONE',  ( -108.7128739231729355, -279.2767854794305435, -286.8350595912751260 ) ) ;
#78944=CARTESIAN_POINT ( 'NONE',  ( 36.48463492266933628, -289.3712653640114354, -256.2295688029942085 ) ) ;
#78946=CARTESIAN_POINT ( 'NONE',  ( 115.2448031289451222, -299.5541904835127980, -192.4725777504219764 ) ) ;
#78947=CARTESIAN_POINT ( 'NONE',  ( 30.87518737893181964, -295.0464627211969741, -237.7469852750401174 ) ) ;
#78949=CARTESIAN_POINT ( 'NONE',  ( -112.3934048168566449, -276.5486602767667819, -270.6202188770992052 ) ) ;
#78950=CARTESIAN_POINT ( 'NONE',  ( -113.2022639796064283, -289.5961707772405589, -282.5813337224485622 ) ) ;
#78951=CARTESIAN_POINT ( 'NONE',  ( -35.65251099251693034, -293.4305128756887484, -344.1544198635715475 ) ) ;
#78952=CARTESIAN_POINT ( 'NONE',  ( -19.39804725191485346, -278.9725256703936793, -199.0394823117002261 ) ) ;
#78953=CARTESIAN_POINT ( 'NONE',  ( -105.6924020575499981, -271.0221210805106580, -240.7433747872985350 ) ) ;
#78954=CARTESIAN_POINT ( 'NONE',  ( -47.07625192294526784, -293.2410892646867637, -197.5155142810987172 ) ) ;
#78955=CARTESIAN_POINT ( 'NONE',  ( 35.78497577281001440, -278.2662352645559167, -287.0191576251351080 ) ) ;
#78956=CARTESIAN_POINT ( 'NONE',  ( -88.15826690957084111, -294.2278172877752240, -327.3563636301191195 ) ) ;
#78957=CARTESIAN_POINT ( 'NONE',  ( -75.10797703767903499, -291.1644666894471811, -333.7806064352284352 ) ) ;
#78958=CARTESIAN_POINT ( 'NONE',  ( -53.15624617916034822, -290.0920747309290846, -195.9845703565227666 ) ) ;
#78959=CARTESIAN_POINT ( 'NONE',  ( 1.638962253470107822, -289.9450202306061897, -332.7781258969576470 ) ) ;
#78961=CARTESIAN_POINT ( 'NONE',  ( -109.9485146625290639, -291.2366339913398292, -279.3529036812778372 ) ) ;
#78963=CARTESIAN_POINT ( 'NONE',  ( -98.89473777838313140, -292.3667677402772824, -224.7405391657489702 ) ) ;
#78964=CARTESIAN_POINT ( 'NONE',  ( 17.97035896663818377, -278.8599975304961163, -219.1851185104262356 ) ) ;
#78965=CARTESIAN_POINT ( 'NONE',  ( -74.97960796736299471, -291.5360538297308608, -207.7530187480938935 ) ) ;
#78966=CARTESIAN_POINT ( 'NONE',  ( -73.75938689446978458, -279.9154809110895030, -202.5265839825511591 ) ) ;
#78967=CARTESIAN_POINT ( 'NONE',  ( 35.58768585597451306, -281.5311615601613653, -295.1651080151920610 ) ) ;
#78968=CARTESIAN_POINT ( 'NONE',  ( 36.24155671752620833, -285.7391356254493644, -284.9361835682964283 ) ) ;
#78970=CARTESIAN_POINT ( 'NONE',  ( 1.731642746028122293, -280.6635912512215327, -333.5411716630344472 ) ) ;
#78971=CARTESIAN_POINT ( 'NONE',  ( -111.0282782149008227, -282.7348430773326982, -256.1168183383626911 ) ) ;
#78972=CARTESIAN_POINT ( 'NONE',  ( -113.5175712458702151, -277.0883914838248074, -265.8952014382018660 ) ) ;
#78973=CARTESIAN_POINT ( 'NONE',  ( -32.31290222346393648, -285.0344713512181443, -193.8221677869262010 ) ) ;
#78974=CARTESIAN_POINT ( 'NONE',  ( -74.36390285328373295, -274.3494877460457815, -207.1996685218972232 ) ) ;
#78976=CARTESIAN_POINT ( 'NONE',  ( -88.49967645557970286, -292.9208466164516835, -217.0992917846135697 ) ) ;
#78977=CARTESIAN_POINT ( 'NONE',  ( 37.33373697168995875, -277.1822559437940185, -286.6144554531836661 ) ) ;
#78978=CARTESIAN_POINT ( 'NONE',  ( -1.463542023603061626, -276.2294975482097357, -334.0174323099013236 ) ) ;
#78979=CARTESIAN_POINT ( 'NONE',  ( -45.27771372789302973, -297.1527124858308184, -344.9919308154136388 ) ) ;
#78980=CARTESIAN_POINT ( 'NONE',  ( -47.74549346304473829, -292.0901649240898905, -194.0134106347832130 ) ) ;
#78981=CARTESIAN_POINT ( 'NONE',  ( 22.61979547779134236, -279.0068178028008674, -224.3624431170859737 ) ) ;
#78982=CARTESIAN_POINT ( 'NONE',  ( 8.852622518109109606, -292.4991279329794907, -208.6903129998639486 ) ) ;
#78983=CARTESIAN_POINT ( 'NONE',  ( -64.14660568663879303, -290.7524386144834807, -202.1939988687319953 ) ) ;
#78984=CARTESIAN_POINT ( 'NONE',  ( -69.96165230614145969, -293.4815471628326691, -337.9099801907603364 ) ) ;
#78987=CARTESIAN_POINT ( 'NONE',  ( -28.09234808330295508, -291.6802321888474125, -197.8366215881910648 ) ) ;
#78989=CARTESIAN_POINT ( 'NONE',  ( 7.450504543161054372, -278.1952119285919025, -214.2458315076590907 ) ) ;
#78990=CARTESIAN_POINT ( 'NONE',  ( -98.09561277386116274, -294.9826697811271288, -317.2842712457926382 ) ) ;
#78991=CARTESIAN_POINT ( 'NONE',  ( -74.02471211983743160, -284.8438110493802355, -337.5592944692355672 ) ) ;
#78992=CARTESIAN_POINT ( 'NONE',  ( 33.02983144176683084, -287.1289582087076155, -250.9485563526661736 ) ) ;
#78993=CARTESIAN_POINT ( 'NONE',  ( 31.91998520578383136, -277.4062370247862646, -295.6794710091879210 ) ) ;
#78994=CARTESIAN_POINT ( 'NONE',  ( 30.98575699803977912, -291.9676829140881296, -300.4144938733773529 ) ) ;
#78995=CARTESIAN_POINT ( 'NONE',  ( -42.43742302147538226, -296.8774444451054819, -344.1988293656959286 ) ) ;
#78997=CARTESIAN_POINT ( 'NONE',  ( 18.60115680843961883, -275.0190396884473785, -317.8745609602932518 ) ) ;
#79000=CARTESIAN_POINT ( 'NONE',  ( -112.2528006584647216, -296.4405859559370242, -252.6390608506351327 ) ) ;
#79001=CARTESIAN_POINT ( 'NONE',  ( 35.42338579777820939, -289.6761622161643004, -286.1231115687391480 ) ) ;
#79002=CARTESIAN_POINT ( 'NONE',  ( -84.44664919488533883, -295.4040081216920726, -211.9331678762224271 ) ) ;
#79003=CARTESIAN_POINT ( 'NONE',  ( 98.49150853115541793, -300.7950733892176913, -193.6458855816779874 ) ) ;
#79004=CARTESIAN_POINT ( 'NONE',  ( 35.73227068942294693, -288.2482951890425511, -273.7563026306463030 ) ) ;
#79005=ORIENTED_EDGE ( 'NONE', *, *, #1254, .F. ) ;
#79006=CARTESIAN_POINT ( 'NONE',  ( -53.69861665899627923, -278.9060841369510513, -195.3049074928894129 ) ) ;
#79007=CARTESIAN_POINT ( 'NONE',  ( -27.75230952064942258, -295.5849626746381773, -346.7121539191600164 ) ) ;
#79008=CARTESIAN_POINT ( 'NONE',  ( -18.06187769216638017, -286.9457734713025161, -343.6318073797739885 ) ) ;
#79009=CARTESIAN_POINT ( 'NONE',  ( -58.84134463458396880, -295.6560185377389871, -344.3322309400725771 ) ) ;
#79011=CARTESIAN_POINT ( 'NONE',  ( 23.35646332321589469, -293.3218543279774622, -229.7677633488392814 ) ) ;
#79016=CARTESIAN_POINT ( 'NONE',  ( 19.75497109296140863, -288.3795467302662132, -219.6602438311696801 ) ) ;
#79017=CARTESIAN_POINT ( 'NONE',  ( -55.63300648810263738, -286.7666405000204577, -350.3538533559490702 ) ) ;
#79018=ORIENTED_EDGE ( 'NONE', *, *, #40970, .F. ) ;
#79020=CARTESIAN_POINT ( 'NONE',  ( -25.40322557732681474, -279.5490952050719784, -194.3954309144580748 ) ) ;
#79021=CARTESIAN_POINT ( 'NONE',  ( -40.28150681293153212, -285.0893599112288825, -345.1366886295930954 ) ) ;
#79022=CARTESIAN_POINT ( 'NONE',  ( -113.7514551305627037, -283.1318528975097024, -269.9666160932473531 ) ) ;
#79023=EDGE_CURVE ( 'NONE', #50851, #89916, #6317, .T. ) ;
#79024=CARTESIAN_POINT ( 'NONE',  ( 36.17763157261016715, -285.7840312171808250, -282.1136053391057885 ) ) ;
#79025=CARTESIAN_POINT ( 'NONE',  ( -28.71772082296576301, -278.8044589720365707, -345.6862236181746084 ) ) ;
#79026=CARTESIAN_POINT ( 'NONE',  ( -110.3630020782395178, -272.9213119432978942, -267.6407032493917768 ) ) ;
#79028=CARTESIAN_POINT ( 'NONE',  ( -68.03742211594335743, -277.4667518209478771, -336.6075814299732087 ) ) ;
#79029=CARTESIAN_POINT ( 'NONE',  ( -94.86593167667261639, -278.5360893408447396, -225.2316014027526023 ) ) ;
#79030=CARTESIAN_POINT ( 'NONE',  ( 28.23108392948699930, -276.1094184174352222, -230.4890014381589367 ) ) ;
#79031=CARTESIAN_POINT ( 'NONE',  ( -113.8135618358849257, -277.4033869928183549, -265.8819345132037597 ) ) ;
#79032=CARTESIAN_POINT ( 'NONE',  ( -71.89434127149799281, -195.1710859107403166, -357.6219360062224268 ) ) ;
#79033=CARTESIAN_POINT ( 'NONE',  ( -71.30950314752216457, -274.5558265749424436, -201.5206606039367045 ) ) ;
#79035=CARTESIAN_POINT ( 'NONE',  ( -95.13742273932719229, -298.6584553923089516, -220.2995219032252123 ) ) ;
#79036=CARTESIAN_POINT ( 'NONE',  ( -110.4542110544635705, -280.8376638359844719, -287.0812184334320705 ) ) ;
#79038=CARTESIAN_POINT ( 'NONE',  ( 82.68005099394714819, -297.1077358065769545, -194.7517231621825147 ) ) ;
#79039=CARTESIAN_POINT ( 'NONE',  ( -74.89019309270882729, -286.6190203524091658, -207.3981387827084291 ) ) ;
#79040=CARTESIAN_POINT ( 'NONE',  ( -112.0068638149089679, -286.4945346981224930, -255.9770754633403556 ) ) ;
#79041=CARTESIAN_POINT ( 'NONE',  ( 34.10854250403009758, -287.1050116826888257, -285.8715098668070596 ) ) ;
#79042=CARTESIAN_POINT ( 'NONE',  ( -92.39408616709890509, -283.3219555224582109, -324.1083197198423136 ) ) ;
#79043=CARTESIAN_POINT ( 'NONE',  ( -11.44352483978653190, -278.7949527497335680, -201.2004479101373988 ) ) ;
#79044=CARTESIAN_POINT ( 'NONE',  ( -30.43964170806274794, -288.0006417698938321, -196.3958146670315443 ) ) ;
#79045=CARTESIAN_POINT ( 'NONE',  ( 24.27276458755230948, -279.4757419249573900, -229.8417711537270236 ) ) ;
#79047=CARTESIAN_POINT ( 'NONE',  ( -32.37058411252477441, -278.3034827085772349, -343.7362568602079591 ) ) ;
#79048=CARTESIAN_POINT ( 'NONE',  ( 35.41586241191881612, -276.1322549328658624, -277.0188604525927758 ) ) ;
#79049=CARTESIAN_POINT ( 'NONE',  ( -17.84029575959824854, -287.6010081967024803, -344.4401564830911298 ) ) ;
#79050=CARTESIAN_POINT ( 'NONE',  ( -18.94712165099068102, -283.6241524709985811, -345.0202402111688116 ) ) ;
#79051=CARTESIAN_POINT ( 'NONE',  ( -76.72100421368769219, -284.0564177298655864, -336.5197632946659496 ) ) ;
#79052=CARTESIAN_POINT ( 'NONE',  ( -35.66492747799724583, -280.2404177230881714, -197.3679749760499931 ) ) ;
#79054=ORIENTED_EDGE ( 'NONE', *, *, #12440, .T. ) ;
#79056=CARTESIAN_POINT ( 'NONE',  ( -3.589367976179181241, -290.4719570152625465, -338.2068158966072815 ) ) ;
#79057=CARTESIAN_POINT ( 'NONE',  ( -111.5123266642346920, -289.4738570064653231, -251.5462952021527769 ) ) ;
#79058=CARTESIAN_POINT ( 'NONE',  ( -68.37139696742067940, -272.6930108850667125, -204.0106120328858879 ) ) ;
#79059=CARTESIAN_POINT ( 'NONE',  ( 4.165289182642732513, -293.8574230422369737, -335.1577442847164434 ) ) ;
#79060=CARTESIAN_POINT ( 'NONE',  ( -31.83871985894098344, -287.4614679239443262, -343.8998055251485084 ) ) ;
#79061=CARTESIAN_POINT ( 'NONE',  ( 35.83646968960238155, -291.9405935366683025, -281.7811788958220518 ) ) ;
#79062=CARTESIAN_POINT ( 'NONE',  ( 19.81478604423949719, -288.1094836800413646, -224.2948569990626879 ) ) ;
#79063=CARTESIAN_POINT ( 'NONE',  ( -106.6379572354042296, -286.6233781216988064, -303.7686719486574702 ) ) ;
#79064=CARTESIAN_POINT ( 'NONE',  ( 33.20028212441003745, -289.8843162594131400, -295.9844924791836434 ) ) ;
#79065=CARTESIAN_POINT ( 'NONE',  ( -110.4847798734278399, -288.3293463769236382, -287.7401912637567420 ) ) ;
#79066=CARTESIAN_POINT ( 'NONE',  ( -69.38839593716652132, -293.6307019692876565, -202.5386052317078907 ) ) ;
#79067=CARTESIAN_POINT ( 'NONE',  ( -95.96145803277369168, -286.1076143495420752, -226.4620014548155780 ) ) ;
#79068=CARTESIAN_POINT ( 'NONE',  ( -1.696263215876659070, -294.5235961217885574, -204.1838465371090763 ) ) ;
#79071=CARTESIAN_POINT ( 'NONE',  ( -108.5558753633842599, -274.8494089183184315, -245.7248023625517703 ) ) ;
#79072=CARTESIAN_POINT ( 'NONE',  ( 21.13281623876076765, -281.3656235168639341, -314.3514955409482354 ) ) ;
#79073=CARTESIAN_POINT ( 'NONE',  ( -37.57154704568068837, -281.0549083849263639, -345.3735404960000892 ) ) ;
#79074=CARTESIAN_POINT ( 'NONE',  ( -66.87185236182260439, -294.6265523897236562, -341.3127909912496989 ) ) ;
#79075=CARTESIAN_POINT ( 'NONE',  ( 18.05875970769074712, -273.0996638547572388, -221.2059969884263353 ) ) ;
#79076=CARTESIAN_POINT ( 'NONE',  ( -109.5752345420029457, -276.3985779199023796, -288.4034757575649337 ) ) ;
#79077=CARTESIAN_POINT ( 'NONE',  ( -77.79732144792812676, -298.8117901221471584, -208.9437320636207858 ) ) ;
#79079=CARTESIAN_POINT ( 'NONE',  ( 34.90629914271126211, -295.1604458767970982, -284.3468793069380354 ) ) ;
#79081=CARTESIAN_POINT ( 'NONE',  ( -61.05586080846941144, -296.1707137011913460, -339.6263701201851291 ) ) ;
#79084=CARTESIAN_POINT ( 'NONE',  ( 37.71877112819517919, -285.4799834931454257, -263.1404935901517206 ) ) ;
#79085=CARTESIAN_POINT ( 'NONE',  ( -86.10028906639864488, -297.3532614223307178, -216.0324882856479007 ) ) ;
#79087=CARTESIAN_POINT ( 'NONE',  ( -95.33473357636955825, -283.8670801881925740, -321.0149240731760187 ) ) ;
#79088=CARTESIAN_POINT ( 'NONE',  ( 38.00368735664729058, -287.0207452104713752, -254.5233471232847364 ) ) ;
#79089=CARTESIAN_POINT ( 'NONE',  ( 5.695741912811828733, -296.4525535926433690, -332.2808796561578788 ) ) ;
#79090=CARTESIAN_POINT ( 'NONE',  ( 37.45454333412241965, -291.5216695783254295, -268.0051919499569522 ) ) ;
#79093=CARTESIAN_POINT ( 'NONE',  ( -71.15430637165700034, -278.8143139629555094, -201.3620855230111886 ) ) ;
#79094=CARTESIAN_POINT ( 'NONE',  ( 21.27581636871891391, -285.6952119285919025, -317.1477375740089997 ) ) ;
#79097=CARTESIAN_POINT ( 'NONE',  ( 9.294548659706796556, -285.5046825457539512, -213.6849254267185074 ) ) ;
#79100=CARTESIAN_POINT ( 'NONE',  ( -103.2559291042665279, -298.5992459676324415, -237.0545789643600756 ) ) ;
#79101=CARTESIAN_POINT ( 'NONE',  ( -45.23072790940431531, -281.3794928385150342, -194.3061017038093041 ) ) ;
#79102=CARTESIAN_POINT ( 'NONE',  ( -97.75827872194228974, -295.1846231798952545, -225.3035629915742390 ) ) ;
#79103=CARTESIAN_POINT ( 'NONE',  ( -18.73563657877088673, -282.8059377833163239, -341.0025749876559757 ) ) ;
#79104=CARTESIAN_POINT ( 'NONE',  ( -93.68802243588953615, -296.0032712453432850, -322.8599799035416709 ) ) ;
#79105=CARTESIAN_POINT ( 'NONE',  ( -44.65699241332127656, -299.4781733326611288, -196.9809026547470978 ) ) ;
#79106=CARTESIAN_POINT ( 'NONE',  ( 24.38317174045481295, -285.0440647485772843, -226.7572176642513568 ) ) ;
#79107=CARTESIAN_POINT ( 'NONE',  ( -95.28887016215765016, -281.2091043488537139, -222.7267916886788157 ) ) ;
#79108=CARTESIAN_POINT ( 'NONE',  ( -98.63795856876178902, -296.1656405682632567, -230.1922296955822560 ) ) ;
#79109=EDGE_LOOP ( 'NONE', ( #15688, #23913 ) ) ;
#79112=CARTESIAN_POINT ( 'NONE',  ( -12.96901330259280094, -284.7139131849630758, -340.9695973012406967 ) ) ;
#79114=CARTESIAN_POINT ( 'NONE',  ( -54.49178911615187104, -292.7666405000204009, -345.3538533559490702 ) ) ;
#79115=CARTESIAN_POINT ( 'NONE',  ( 34.57422617065304138, -274.4062564883361119, -243.3008451689669300 ) ) ;
#79116=CARTESIAN_POINT ( 'NONE',  ( -46.99236405961787000, -291.7594739362023688, -198.0018429020756798 ) ) ;
#79117=CARTESIAN_POINT ( 'NONE',  ( -2.841480226516286400, -282.0369403942364102, -205.2281265122227865 ) ) ;
#79118=CARTESIAN_POINT ( 'NONE',  ( -1.059344518266583934, -278.1625950007542087, -334.6842715454314430 ) ) ;
#79120=CARTESIAN_POINT ( 'NONE',  ( 15.21663046659259777, -283.9248511803010047, -325.5341394619395601 ) ) ;
#79121=CARTESIAN_POINT ( 'NONE',  ( 34.03269716037721082, -280.5722925279946480, -287.5266992562808923 ) ) ;
#79122=CARTESIAN_POINT ( 'NONE',  ( -101.1832053299107486, -281.0817090324558762, -230.9013124160785537 ) ) ;
#79123=CARTESIAN_POINT ( 'NONE',  ( -114.1811869102184005, -272.7905278953037964, -264.6283571190233488 ) ) ;
#79124=CARTESIAN_POINT ( 'NONE',  ( 36.58645825288770936, -275.1133394998580002, -248.6427643975326305 ) ) ;
#79125=CARTESIAN_POINT ( 'NONE',  ( -0.01511613712742478077, -296.4718781068817179, -334.8252405970216046 ) ) ;
#79126=CARTESIAN_POINT ( 'NONE',  ( 82.64890176555634582, -299.5541904835127980, -195.3611179825600175 ) ) ;
#79128=CARTESIAN_POINT ( 'NONE',  ( -1.314739369625168353, -292.7191797656094536, -337.0268208193561463 ) ) ;
#79129=CARTESIAN_POINT ( 'NONE',  ( 7.373518244478687755, -274.1886147104881388, -212.5810376143959957 ) ) ;
#79130=CARTESIAN_POINT ( 'NONE',  ( -50.46630693259032086, -293.4075994641766556, -195.1916265162254831 ) ) ;
#79131=CARTESIAN_POINT ( 'NONE',  ( -47.70494487000384254, -293.1283933619608888, -194.4089047197740001 ) ) ;
#79132=CARTESIAN_POINT ( 'NONE',  ( -71.99977451636554804, -291.5116069859776644, -336.6993920046007815 ) ) ;
#79133=CARTESIAN_POINT ( 'NONE',  ( -98.39585236367773291, -275.9623592486655070, -313.6548391610912745 ) ) ;
#79134=CARTESIAN_POINT ( 'NONE',  ( -74.71551201268076170, -279.4739139996365793, -334.7390053621615493 ) ) ;
#79135=CARTESIAN_POINT ( 'NONE',  ( 34.70801452054603686, -291.3897363786066990, -251.6487472191906818 ) ) ;
#79136=CARTESIAN_POINT ( 'NONE',  ( 5.466522107261644337, -282.4854320657289009, -207.8490264524213273 ) ) ;
#79137=CARTESIAN_POINT ( 'NONE',  ( -25.07662646889796676, -285.1324192832180415, -198.0337823598655120 ) ) ;
#79139=CARTESIAN_POINT ( 'NONE',  ( -70.22824800684831814, -283.1646185734084611, -335.5714386945235788 ) ) ;
#79140=CARTESIAN_POINT ( 'NONE',  ( -48.08911779156115074, -280.9982872853623803, -194.3734018237312853 ) ) ;
#79142=CARTESIAN_POINT ( 'NONE',  ( -83.02670602741321204, -284.2376725254912344, -208.8060475509723517 ) ) ;
#79143=CARTESIAN_POINT ( 'NONE',  ( -113.9766550460613388, -279.5493691389406195, -265.8997395984927721 ) ) ;
#79145=CARTESIAN_POINT ( 'NONE',  ( -35.70678016555273615, -278.5521401201835374, -346.6632756690524957 ) ) ;
#79146=CARTESIAN_POINT ( 'NONE',  ( -67.74223827176244583, -300.1233781216987495, -207.3071070584150277 ) ) ;
#79149=CARTESIAN_POINT ( 'NONE',  ( -87.45505899282771622, -299.3530998756441477, -214.5610112669792784 ) ) ;
#79151=CARTESIAN_POINT ( 'NONE',  ( -110.7450684565213237, -276.7471581634047766, -256.8041152558170666 ) ) ;
#79152=CARTESIAN_POINT ( 'NONE',  ( -92.09764668828397305, -293.0437876989532811, -217.6007511112921975 ) ) ;
#79153=CARTESIAN_POINT ( 'NONE',  ( 31.63347452782329938, -293.2242548381822189, -294.7266388817492384 ) ) ;
#79154=CARTESIAN_POINT ( 'NONE',  ( -111.8639968354835759, -289.8196206036510034, -289.5437691581154240 ) ) ;
#79156=CARTESIAN_POINT ( 'NONE',  ( 37.77463523503917031, -292.3042784182760556, -284.4368143448964474 ) ) ;
#79157=CARTESIAN_POINT ( 'NONE',  ( -92.10128173253971795, -283.6536421092041564, -220.8105176714796301 ) ) ;
#79158=CARTESIAN_POINT ( 'NONE',  ( -36.21068021588382635, -293.9268608346539509, -196.1218426852248911 ) ) ;
#79159=CARTESIAN_POINT ( 'NONE',  ( 15.54038276650088335, -285.2969932414598588, -219.0367274753635058 ) ) ;
#79160=CARTESIAN_POINT ( 'NONE',  ( -59.07811424488186702, -284.6544381370603105, -340.6198266281787710 ) ) ;
#79161=CARTESIAN_POINT ( 'NONE',  ( -48.82193415238505452, -290.1360675601515595, -346.3163090201454111 ) ) ;
#79163=CARTESIAN_POINT ( 'NONE',  ( 7.174861181162916601, -281.1694834442748743, -212.3638368555477598 ) ) ;
#79164=CARTESIAN_POINT ( 'NONE',  ( 35.10584442259728633, -292.6642061806714423, -295.4105569810564020 ) ) ;
#79165=CARTESIAN_POINT ( 'NONE',  ( -62.70069236034566984, -290.1766794308061321, -342.9506861697240652 ) ) ;
#79166=CARTESIAN_POINT ( 'NONE',  ( -111.4809927416646786, -290.7866492086951666, -290.9254607659004250 ) ) ;
#79167=CARTESIAN_POINT ( 'NONE',  ( -107.3555660689203535, -284.9943675809792580, -249.5203869174166016 ) ) ;
#79170=CARTESIAN_POINT ( 'NONE',  ( 10.43801928303763304, -296.2614184942102042, -329.2284366008932466 ) ) ;
#79172=CARTESIAN_POINT ( 'NONE',  ( -83.89846522891659220, -294.3610253939189079, -331.1384331895002902 ) ) ;
#79174=CARTESIAN_POINT ( 'NONE',  ( -103.5775531740153070, -278.0331414421972340, -238.9974402746694579 ) ) ;
#79175=CARTESIAN_POINT ( 'NONE',  ( -102.6634798842978853, -272.5920660887801432, -229.7090332559016019 ) ) ;
#79176=CARTESIAN_POINT ( 'NONE',  ( -96.16939046213497022, -294.4141897305299267, -314.7667137625541613 ) ) ;
#79177=CARTESIAN_POINT ( 'NONE',  ( 7.933341928168413659, -276.4407406380216230, -211.8107586522377517 ) ) ;
#79178=CARTESIAN_POINT ( 'NONE',  ( -72.47168884725178373, -271.7219804956460507, -204.9069881082111806 ) ) ;
#79179=CARTESIAN_POINT ( 'NONE',  ( 34.33426082907095633, -294.5491481207010906, -254.5015656391188088 ) ) ;
#79180=CARTESIAN_POINT ( 'NONE',  ( -42.39737519490049067, -296.1970844667483789, -343.4956940975026214 ) ) ;
#79183=CARTESIAN_POINT ( 'NONE',  ( -104.8552138059868355, -294.9866993970192652, -237.3163923170674536 ) ) ;
#79184=CARTESIAN_POINT ( 'NONE',  ( -78.15539735354644790, -298.1699746117717496, -205.1878496493273758 ) ) ;
#79185=CARTESIAN_POINT ( 'NONE',  ( 34.27032864867291551, -286.3486184444865899, -287.3049148862441484 ) ) ;
#79186=CARTESIAN_POINT ( 'NONE',  ( -108.2041732384576136, -274.8703032238392439, -245.7946662149102508 ) ) ;
#79187=CARTESIAN_POINT ( 'NONE',  ( -82.68258255700632731, -290.6308873868062506, -327.8729674393077289 ) ) ;
#79188=CARTESIAN_POINT ( 'NONE',  ( -41.19596605583647886, -274.4973417007616945, -193.4670396566185389 ) ) ;
#79189=CARTESIAN_POINT ( 'NONE',  ( -86.11756378033236103, -297.6864889449599332, -216.0195812756013254 ) ) ;
#79190=CARTESIAN_POINT ( 'NONE',  ( -107.1235865821047923, -280.1629335888137007, -298.8021995940503643 ) ) ;
#79191=CARTESIAN_POINT ( 'NONE',  ( -5.136241568587593065, -279.1521010794865560, -200.9629428362322301 ) ) ;
#79192=VECTOR ( 'NONE', #36946, 1000.000000000000000 ) ;
#79194=CARTESIAN_POINT ( 'NONE',  ( -10.74508538605319252, -282.0629559478086890, -342.5698375703375405 ) ) ;
#79195=CARTESIAN_POINT ( 'NONE',  ( 37.18848437168953325, -274.6634824389688561, -251.4253215798912890 ) ) ;
#79196=CARTESIAN_POINT ( 'NONE',  ( -112.4445264367236206, -277.1148561300767028, -257.4767904211815903 ) ) ;
#79197=CARTESIAN_POINT ( 'NONE',  ( -91.72920324885171794, -277.2794066225720826, -218.4020228094826166 ) ) ;
#79198=CARTESIAN_POINT ( 'NONE',  ( -82.23219027768399769, -296.1101563351843424, -212.1065338035345462 ) ) ;
#79199=CARTESIAN_POINT ( 'NONE',  ( 22.14554948011263136, -278.1781031353681897, -316.0573655045046735 ) ) ;
#79201=CARTESIAN_POINT ( 'NONE',  ( -63.78743207815339389, -289.7293003644548435, -199.7439107473451543 ) ) ;
#79202=CARTESIAN_POINT ( 'NONE',  ( -108.3671355284131153, -290.9304081750996716, -240.6224642438094179 ) ) ;
#79203=CARTESIAN_POINT ( 'NONE',  ( -30.04286117087120545, -276.1444902713843703, -195.5496524448937237 ) ) ;
#79204=CARTESIAN_POINT ( 'NONE',  ( 10.41666703503159752, -296.6511620856778109, -195.5441041681855836 ) ) ;
#79205=CARTESIAN_POINT ( 'NONE',  ( -36.55679133239928547, -285.2589399554745455, -193.5135908881578359 ) ) ;
#79207=CARTESIAN_POINT ( 'NONE',  ( -109.9508466224932448, -282.3100271914942141, -289.1971549417632446 ) ) ;
#79209=CARTESIAN_POINT ( 'NONE',  ( 18.79011748054693953, -291.6788726799870233, -223.0710602766620525 ) ) ;
#79210=CARTESIAN_POINT ( 'NONE',  ( -27.65226149678700196, -284.3161051638186336, -196.7609803617324644 ) ) ;
#79213=CARTESIAN_POINT ( 'NONE',  ( -38.39525521212431869, -293.0652040535756555, -345.3537221148486083 ) ) ;
#79214=CARTESIAN_POINT ( 'NONE',  ( -110.0310385852859412, -282.7370229505635848, -293.6199233642132640 ) ) ;
#79215=CARTESIAN_POINT ( 'NONE',  ( -92.82318459905957297, -280.8394905825547312, -221.6772668069955898 ) ) ;
#79216=CARTESIAN_POINT ( 'NONE',  ( -112.1340618130393381, -285.5490890516229570, -286.9174265703881588 ) ) ;
#79217=CARTESIAN_POINT ( 'NONE',  ( -11.82819930766667937, -278.6195267798581767, -198.7304837180949733 ) ) ;
#79218=CARTESIAN_POINT ( 'NONE',  ( 29.96176989014811198, -287.1712389254042819, -241.9593260917929740 ) ) ;
#79219=CARTESIAN_POINT ( 'NONE',  ( -74.29357734612666775, -278.9791120927117731, -334.0002072866249136 ) ) ;
#79220=CARTESIAN_POINT ( 'NONE',  ( -85.59834137066741278, -280.1668156007853554, -215.3711343266621441 ) ) ;
#79221=CARTESIAN_POINT ( 'NONE',  ( 1.863285120913890758, -288.5538547089687995, -206.0075948949304063 ) ) ;
#79224=CARTESIAN_POINT ( 'NONE',  ( -87.46065125704886611, -297.2089218747166797, -211.8349436728260571 ) ) ;
#79225=CARTESIAN_POINT ( 'NONE',  ( 37.30014109282085855, -289.5406304514935982, -271.0262034806245310 ) ) ;
#79226=DIRECTION ( 'NONE',  ( 0.9951408606192336803, 1.205805641958489930E-17, 0.09846150276128748380 ) ) ;
#79227=CARTESIAN_POINT ( 'NONE',  ( 36.57525178469696669, -283.6233781216987495, -234.7283546768995564 ) ) ;
#79228=ORIENTED_EDGE ( 'NONE', *, *, #60782, .T. ) ;
#79229=CARTESIAN_POINT ( 'NONE',  ( -10.96646584678391179, -272.3948899111013588, -199.9184127489230889 ) ) ;
#79230=CARTESIAN_POINT ( 'NONE',  ( 30.19937651941408419, -291.4908078802423574, -234.9679656265668939 ) ) ;
#79231=VECTOR ( 'NONE', #57318, 1000.000000000000000 ) ;
#79232=CARTESIAN_POINT ( 'NONE',  ( 35.20763525599286226, -289.2413003401826472, -283.2956333914979723 ) ) ;
#79233=CARTESIAN_POINT ( 'NONE',  ( 21.30532312359792968, -282.6853001640905063, -225.1907700664478114 ) ) ;
#79234=CARTESIAN_POINT ( 'NONE',  ( 32.16840943306019796, -288.5671842924766111, -238.5013208956435449 ) ) ;
#79235=CARTESIAN_POINT ( 'NONE',  ( 35.48350285086903000, -289.1640813842440707, -293.8086782746200356 ) ) ;
#79236=CARTESIAN_POINT ( 'NONE',  ( -111.9875524087367467, -286.6523929854164408, -262.5668472399709117 ) ) ;
#79237=CARTESIAN_POINT ( 'NONE',  ( -104.9745736888721126, -278.2425155916996005, -307.1686500703929141 ) ) ;
#79239=CARTESIAN_POINT ( 'NONE',  ( 37.18190053272848417, -291.7919480627124926, -282.9112189660622221 ) ) ;
#79240=CARTESIAN_POINT ( 'NONE',  ( 22.87664135533223231, -280.7427912518157882, -222.3531636890328969 ) ) ;
#79242=CARTESIAN_POINT ( 'NONE',  ( -81.82987380639806929, -275.2996919761560548, -210.8687624162998588 ) ) ;
#79243=CARTESIAN_POINT ( 'NONE',  ( 35.78497577281001440, -284.2662352645559167, -287.0191576251351080 ) ) ;
#79244=CARTESIAN_POINT ( 'NONE',  ( -8.060068942809543557, -272.6701934210207128, -200.1870704116645925 ) ) ;
#79246=CARTESIAN_POINT ( 'NONE',  ( -79.08489616690248170, -278.9795500921525218, -210.3986795233574298 ) ) ;
#79248=CARTESIAN_POINT ( 'NONE',  ( 10.29121740237822813, -277.6169604270226614, -330.4214784075297757 ) ) ;
#79249=CARTESIAN_POINT ( 'NONE',  ( -84.46597058586647222, -298.8141453474012224, -213.7730891900556571 ) ) ;
#79250=CARTESIAN_POINT ( 'NONE',  ( -111.2681219997007815, -283.3509651492554440, -291.0421325272392323 ) ) ;
#79251=CARTESIAN_POINT ( 'NONE',  ( -111.2590721523700523, -292.3730280653362570, -265.6937478498151677 ) ) ;
#79252=CARTESIAN_POINT ( 'NONE',  ( -89.62888855191683035, -274.9301236646655298, -214.8589935751236339 ) ) ;
#79253=CARTESIAN_POINT ( 'NONE',  ( -101.2270568954744334, -298.3163578548013106, -228.0682072674906635 ) ) ;
#79254=CARTESIAN_POINT ( 'NONE',  ( 35.23007647460011071, -295.7873720894159533, -288.6194221403023903 ) ) ;
#79255=CARTESIAN_POINT ( 'NONE',  ( -64.74997717118750984, -281.4107401076751671, -339.9945494405054660 ) ) ;
#79256=CARTESIAN_POINT ( 'NONE',  ( -112.6183988753795262, -290.4210039483884316, -254.2004064992852079 ) ) ;
#79257=CARTESIAN_POINT ( 'NONE',  ( -13.51712384418907220, -272.3831178840140979, -199.6204905742507663 ) ) ;
#79258=CARTESIAN_POINT ( 'NONE',  ( 11.54852554760831751, -288.3171162900156901, -211.8441302997285334 ) ) ;
#79260=CARTESIAN_POINT ( 'NONE',  ( -90.02896461324502297, -290.2059925061471404, -219.3878089412581858 ) ) ;
#79262=CARTESIAN_POINT ( 'NONE',  ( -113.5986427952308162, -289.1879564377489942, -265.5149868868106751 ) ) ;
#79263=CARTESIAN_POINT ( 'NONE',  ( 29.44267672351397991, -287.6176442639592210, -300.0150900073157914 ) ) ;
#79265=CARTESIAN_POINT ( 'NONE',  ( -36.58235796575990406, -287.1411389333542843, -193.6610016213380732 ) ) ;
#79266=CARTESIAN_POINT ( 'NONE',  ( -71.66036869292177869, -277.8520523299818592, -334.8292086342329981 ) ) ;
#79267=CARTESIAN_POINT ( 'NONE',  ( 21.97893736620609317, -291.8171726277817584, -221.7550023347215529 ) ) ;
#79268=CARTESIAN_POINT ( 'NONE',  ( -111.0079393896297830, -284.9258550523901476, -292.4657919527791705 ) ) ;
#79270=CARTESIAN_POINT ( 'NONE',  ( -73.60680702994881131, -285.9179544681879861, -202.4007802720128950 ) ) ;
#79271=CARTESIAN_POINT ( 'NONE',  ( -54.50187413213997445, -280.1589559689548992, -199.3327404989723561 ) ) ;
#79272=CARTESIAN_POINT ( 'NONE',  ( 168.3298383987194882, 232.4948596809232981, -192.7828393143454662 ) ) ;
#79273=CARTESIAN_POINT ( 'NONE',  ( -104.9900673867532390, -255.0990985645446472, -326.1467328686887868 ) ) ;
#79274=CARTESIAN_POINT ( 'NONE',  ( -107.0431942798137328, -259.6916240115564278, -315.7347989823788907 ) ) ;
#79275=CARTESIAN_POINT ( 'NONE',  ( -32.67053191954658331, -273.3096596052347422, -197.3363601573703932 ) ) ;
#79276=CARTESIAN_POINT ( 'NONE',  ( 31.41297026965077066, -274.1347254352875780, -244.9245031990116956 ) ) ;
#79277=CARTESIAN_POINT ( 'NONE',  ( -27.76171907815665563, -294.4413865408643574, -346.7540745993601945 ) ) ;
#79278=CARTESIAN_POINT ( 'NONE',  ( -110.4136115702177534, -272.0207119292052766, -270.3543514753225168 ) ) ;
#79279=CARTESIAN_POINT ( 'NONE',  ( -57.97242737162893889, -272.4760277047526529, -196.6333199867409860 ) ) ;
#79280=CARTESIAN_POINT ( 'NONE',  ( -96.28402587452860928, -299.0370821061700326, -225.2109424934774324 ) ) ;
#79281=CARTESIAN_POINT ( 'NONE',  ( 36.12372930229673784, -288.9119491651757698, -273.7660875163248306 ) ) ;
#79283=CARTESIAN_POINT ( 'NONE',  ( -113.7079270744290085, -297.3954088188022524, -278.1726219702486560 ) ) ;
#79284=CARTESIAN_POINT ( 'NONE',  ( 22.03793322046877989, -287.4489908733972925, -227.7076796636168297 ) ) ;
#79285=CARTESIAN_POINT ( 'NONE',  ( -89.94081171471141545, -272.2507554532513154, -214.4779847718323822 ) ) ;
#79286=CARTESIAN_POINT ( 'NONE',  ( 36.54606754633113042, -294.0895197576217583, -249.2239446446268687 ) ) ;
#79287=CARTESIAN_POINT ( 'NONE',  ( -79.43804899968603195, -296.0967265333636647, -334.7616173191334497 ) ) ;
#79288=CARTESIAN_POINT ( 'NONE',  ( -37.55208115942573954, -292.2161625842783224, -197.3489774290588059 ) ) ;
#79290=CARTESIAN_POINT ( 'NONE',  ( 1.653509048599000053, -276.4894406914506249, -205.6410449075851830 ) ) ;
#79291=CARTESIAN_POINT ( 'NONE',  ( 37.20189734825071781, -274.5695240603387219, -288.0601536754574568 ) ) ;
#79293=ORIENTED_EDGE ( 'NONE', *, *, #68252, .F. ) ;
#79294=CARTESIAN_POINT ( 'NONE',  ( -95.85492304601467595, -278.7343735814407637, -220.3836064735843649 ) ) ;
#79295=CARTESIAN_POINT ( 'NONE',  ( 34.61832745809518741, -273.7376640446825036, -253.9278914373810494 ) ) ;
#79296=CARTESIAN_POINT ( 'NONE',  ( -39.19364753710746641, -299.2335101995858508, -196.9749353761709472 ) ) ;
#79298=CARTESIAN_POINT ( 'NONE',  ( 3.049753577997755372, -275.5501753835582690, -209.2109191504288788 ) ) ;
#79299=CARTESIAN_POINT ( 'NONE',  ( 21.95335451253598436, -276.6670157383317701, -222.8213331975953224 ) ) ;
#79300=CARTESIAN_POINT ( 'NONE',  ( -5.992532915547622352, -274.6622623917905912, -338.8858326596716211 ) ) ;
#79301=CARTESIAN_POINT ( 'NONE',  ( -10.44478960713967730, -295.3430996826278943, -338.3350017373052765 ) ) ;
#79302=CARTESIAN_POINT ( 'NONE',  ( 18.40703316846486715, -292.8057323675732277, -318.4162873627262229 ) ) ;
#79304=CARTESIAN_POINT ( 'NONE',  ( -113.7043659784540779, -278.9216275648375927, -280.1778724609583264 ) ) ;
#79305=CARTESIAN_POINT ( 'NONE',  ( -7.505709589569036666, -276.8163995321488642, -336.9855404799735084 ) ) ;
#79307=CARTESIAN_POINT ( 'NONE',  ( -7.519800223873003731, -285.1197312858404302, -199.8494956847380877 ) ) ;
#79308=CARTESIAN_POINT ( 'NONE',  ( -110.8077760466121617, -298.3486259274380359, -286.2596751496527645 ) ) ;
#79309=CARTESIAN_POINT ( 'NONE',  ( 82.61719680589260406, -302.0442921925621818, -195.6390021813133160 ) ) ;
#79311=CARTESIAN_POINT ( 'NONE',  ( 34.44060564382931489, -286.9362699305750084, -284.5645155065549261 ) ) ;
#79313=CARTESIAN_POINT ( 'NONE',  ( -73.35440364028322335, -275.7765358487981757, -335.0368119225725536 ) ) ;
#79314=CARTESIAN_POINT ( 'NONE',  ( -70.73628142453387113, -276.0763636839209312, -335.9368517470212510 ) ) ;
#79315=CARTESIAN_POINT ( 'NONE',  ( 2.749136002822625269, -284.5149216349033736, -333.8072594197521994 ) ) ;
#79316=CARTESIAN_POINT ( 'NONE',  ( -24.24375094371539063, -278.0864058131802494, -342.6317827543850854 ) ) ;
#79318=AXIS2_PLACEMENT_3D ( 'NONE', #63011, #4742, #69613 ) ;
#79319=CARTESIAN_POINT ( 'NONE',  ( 13.44660569223658797, -273.1485362273969599, -213.4840009222043875 ) ) ;
#79320=CARTESIAN_POINT ( 'NONE',  ( 35.80096514414278630, -276.2196051627906854, -271.5783972681992395 ) ) ;
#79321=CARTESIAN_POINT ( 'NONE',  ( 10.34954366717665408, -284.3963923765912227, -328.5281780728930698 ) ) ;
#79323=CARTESIAN_POINT ( 'NONE',  ( -12.67036102426736299, -290.6541716096697883, -341.8347116628407321 ) ) ;
#79324=CARTESIAN_POINT ( 'NONE',  ( 25.67196727737569972, -291.0028610460252025, -229.5940249424465947 ) ) ;
#79327=CARTESIAN_POINT ( 'NONE',  ( -105.8700488886609321, -271.5910814826529531, -243.6669348667808492 ) ) ;
#79328=CARTESIAN_POINT ( 'NONE',  ( 9.648728131138632591, -290.8458101595338690, -212.8247370813005830 ) ) ;
#79329=CARTESIAN_POINT ( 'NONE',  ( -71.74250447947856912, -195.9422791308210492, -360.7315132586310824 ) ) ;
#79331=CARTESIAN_POINT ( 'NONE',  ( -99.31855673999471890, -288.4364252299862983, -314.8984196397925643 ) ) ;
#79332=CARTESIAN_POINT ( 'NONE',  ( -106.9212331156635827, -285.8266585589992133, -295.1125431093550446 ) ) ;
#79333=CARTESIAN_POINT ( 'NONE',  ( -111.5405219295187322, -282.5843521073865077, -286.7473579667551462 ) ) ;
#79335=CARTESIAN_POINT ( 'NONE',  ( -26.63928815698761454, -284.3387630025928274, -343.2196550639237671 ) ) ;
#79336=CARTESIAN_POINT ( 'NONE',  ( -107.5439860226457682, -285.0825507067057742, -291.0029320709091962 ) ) ;
#79337=CARTESIAN_POINT ( 'NONE',  ( -112.5479154642533075, -292.5925726325560845, -265.6248773695701857 ) ) ;
#79338=CARTESIAN_POINT ( 'NONE',  ( 24.46036004656913576, -275.2750418548525886, -224.4672224215528900 ) ) ;
#79339=CARTESIAN_POINT ( 'NONE',  ( -109.0562938438775973, -288.9391456062112979, -246.3998300853839680 ) ) ;
#79340=CARTESIAN_POINT ( 'NONE',  ( -48.49398732360806008, -277.1902394656632964, -346.6031117644668598 ) ) ;
#79341=CARTESIAN_POINT ( 'NONE',  ( 34.19837377620675767, -295.2542288733499163, -248.8791137200036019 ) ) ;
#79344=CARTESIAN_POINT ( 'NONE',  ( -110.8125350698461062, -283.1939605091968133, -273.6435707378785764 ) ) ;
#79345=CARTESIAN_POINT ( 'NONE',  ( 7.375061520024341455, -278.6611978120652680, -210.0851517577858090 ) ) ;
#79346=CARTESIAN_POINT ( 'NONE',  ( -26.33290810456523801, -296.5876796138260829, -194.1640512332339767 ) ) ;
#79347=CARTESIAN_POINT ( 'NONE',  ( 29.18224716367678084, -274.4912446551933272, -239.9325772984570904 ) ) ;
#79348=CARTESIAN_POINT ( 'NONE',  ( 28.09337909425091340, -294.6156375422528413, -236.4648326735461694 ) ) ;
#79349=CARTESIAN_POINT ( 'NONE',  ( 35.52818187999859134, -294.3908957125574375, -262.5649926542702133 ) ) ;
#79350=CARTESIAN_POINT ( 'NONE',  ( 10.90041765718997091, -295.7162643014032142, -329.8095014548617314 ) ) ;
#79351=CARTESIAN_POINT ( 'NONE',  ( -77.95150399151039267, -295.4477271009009200, -331.0838915039066137 ) ) ;
#79352=CARTESIAN_POINT ( 'NONE',  ( -108.8515009288287700, -292.2585448295339461, -293.1457307293347867 ) ) ;
#79353=CARTESIAN_POINT ( 'NONE',  ( -47.25425948742065430, -283.3414768375047288, -346.7204079965562755 ) ) ;
#79354=CARTESIAN_POINT ( 'NONE',  ( 6.539205181120335553, -272.7806781962858054, -208.5328814618266620 ) ) ;
#79355=CARTESIAN_POINT ( 'NONE',  ( 33.86023690505374617, -287.0113946112132339, -240.9082656323979279 ) ) ;
#79356=CARTESIAN_POINT ( 'NONE',  ( -111.1138814072980949, -280.3852289015279666, -281.7414550896880314 ) ) ;
#79358=CARTESIAN_POINT ( 'NONE',  ( -9.392535180193947397, -285.4853726225501305, -202.6552273925655356 ) ) ;
#79359=CARTESIAN_POINT ( 'NONE',  ( -68.54896417137751996, -287.4620365862920721, -338.5741968564388458 ) ) ;
#79360=CARTESIAN_POINT ( 'NONE',  ( -94.07136297056315755, -227.2831051785662737, -345.8935872616412439 ) ) ;
#79361=CARTESIAN_POINT ( 'NONE',  ( -108.7236849902738811, -284.2658687704948761, -254.7270880068594465 ) ) ;
#79362=CARTESIAN_POINT ( 'NONE',  ( 38.48044124476435002, -282.8943667953496970, -281.2703615932797447 ) ) ;
#79363=CARTESIAN_POINT ( 'NONE',  ( -15.03212033496614453, -287.8289575683895123, -343.8680599547374186 ) ) ;
#79364=CARTESIAN_POINT ( 'NONE',  ( -112.9262887534446804, -280.2795032123980832, -260.2939720749303660 ) ) ;
#79365=CARTESIAN_POINT ( 'NONE',  ( -103.1728610879883519, -279.3550290190643750, -309.4464600763727162 ) ) ;
#79366=CARTESIAN_POINT ( 'NONE',  ( -4.345669664768961660, -280.3329431615647422, -205.2299327592702127 ) ) ;
#79367=CARTESIAN_POINT ( 'NONE',  ( 14.62405027875340835, -276.7680307453410933, -216.7756014152288060 ) ) ;
#79368=CARTESIAN_POINT ( 'NONE',  ( 17.48960558643630492, -292.8090164105687450, -216.2256281858508657 ) ) ;
#79369=CARTESIAN_POINT ( 'NONE',  ( 32.93976373489518750, -285.8997161556771403, -295.5079396244279906 ) ) ;
#79370=CARTESIAN_POINT ( 'NONE',  ( -95.97647708291485458, -292.8136972994762459, -221.6747022778889118 ) ) ;
#79371=CARTESIAN_POINT ( 'NONE',  ( -100.4395064246689344, -294.9606411727545492, -307.7825840145277425 ) ) ;
#79372=CARTESIAN_POINT ( 'NONE',  ( -21.04970008677109661, -284.7617937203186216, -343.0494474300388106 ) ) ;
#79373=CARTESIAN_POINT ( 'NONE',  ( -61.02403558633059077, -295.0347830011712063, -339.4888322163977818 ) ) ;
#79374=CARTESIAN_POINT ( 'NONE',  ( -61.60387747519136070, -292.8239548325258852, -197.5532807902221180 ) ) ;
#79375=TOROIDAL_SURFACE ( 'NONE', #62762, 5.654241149514405151, 1.000000000000000000 ) ;
#79376=CARTESIAN_POINT ( 'NONE',  ( 34.16316661659890741, -282.0026176563101785, -255.1045770131308927 ) ) ;
#79377=CARTESIAN_POINT ( 'NONE',  ( -68.73683545235036263, -272.7082355036955619, -200.2956032055256514 ) ) ;
#79378=CARTESIAN_POINT ( 'NONE',  ( -14.97396002511934299, -289.4213663311979303, -343.9898697297467720 ) ) ;
#79379=CARTESIAN_POINT ( 'NONE',  ( -69.96016351343914152, -281.6167039092179039, -338.7591289979116596 ) ) ;
#79380=CARTESIAN_POINT ( 'NONE',  ( -87.36747178958346183, -290.0606781802754881, -328.9389609374773613 ) ) ;
#79381=CARTESIAN_POINT ( 'NONE',  ( 16.90347899137946186, -287.1855028478344138, -221.4594488146300080 ) ) ;
#79382=CARTESIAN_POINT ( 'NONE',  ( 195.3599902543797953, 284.4457220976750023, -111.0290403122453853 ) ) ;
#79383=CARTESIAN_POINT ( 'NONE',  ( -47.65177483170455019, -155.1274943976620193, -361.2761651912329626 ) ) ;
#79385=CARTESIAN_POINT ( 'NONE',  ( -104.5864771384207188, -278.1356585658369340, -241.5385280345304579 ) ) ;
#79386=CARTESIAN_POINT ( 'NONE',  ( -36.99311476855296377, -278.9769453226023188, -197.0528335737728298 ) ) ;
#79387=CARTESIAN_POINT ( 'NONE',  ( -5.119248141194297830, -274.1315397973618246, -200.4507619572238752 ) ) ;
#79388=CARTESIAN_POINT ( 'NONE',  ( 104.7727649842400837, 114.2745951806146110, -280.7604989259197623 ) ) ;
#79389=CARTESIAN_POINT ( 'NONE',  ( -109.0469055283881517, -277.4648587663873514, -243.8082740606749894 ) ) ;
#79390=CARTESIAN_POINT ( 'NONE',  ( -21.05331540121727230, -280.8623749884079643, -343.2602689546508259 ) ) ;
#79391=CARTESIAN_POINT ( 'NONE',  ( -113.3248995114598188, -298.3214972268601173, -269.6348792102214702 ) ) ;
#79393=CARTESIAN_POINT ( 'NONE',  ( -103.6147698734461642, -291.4592933310277658, -239.6061400442966374 ) ) ;
#79394=CARTESIAN_POINT ( 'NONE',  ( -64.01539613199562950, -288.0921720306158136, -338.8974781640059177 ) ) ;
#79395=CARTESIAN_POINT ( 'NONE',  ( 28.41107721460962665, -275.6812292215259390, -230.3859765899375986 ) ) ;
#79396=CARTESIAN_POINT ( 'NONE',  ( 94.40783104291642758, -299.9133832367027139, -197.3573954632416019 ) ) ;
#79400=CARTESIAN_POINT ( 'NONE',  ( -64.25276690779156752, -281.6240354246907032, -199.7006295994097513 ) ) ;
#79401=CARTESIAN_POINT ( 'NONE',  ( 33.40830374475189757, -282.3786859598549199, -251.1125251686990794 ) ) ;
#79402=CARTESIAN_POINT ( 'NONE',  ( 19.35742575148746880, -282.6170543035222522, -219.7531905657830009 ) ) ;
#79403=CARTESIAN_POINT ( 'NONE',  ( -87.09745701662976103, -282.8241301725437893, -324.1685124379164904 ) ) ;
#79404=CARTESIAN_POINT ( 'NONE',  ( -101.6410646100322879, -279.9110861967631081, -307.5649388899048517 ) ) ;
#79405=CARTESIAN_POINT ( 'NONE',  ( 17.81726478191379925, -273.3396443488283580, -221.4163044101814251 ) ) ;
#79408=CARTESIAN_POINT ( 'NONE',  ( -39.94721566163005377, -277.8869032648578923, -347.1684933255999113 ) ) ;
#79411=CARTESIAN_POINT ( 'NONE',  ( -45.60408299473439087, -275.7295098113027052, -346.3765204302799248 ) ) ;
#79412=ORIENTED_EDGE ( 'NONE', *, *, #80614, .F. ) ;
#79414=CARTESIAN_POINT ( 'NONE',  ( -82.86897144359556933, -285.6508145197346948, -330.4739166430243813 ) ) ;
#79415=CARTESIAN_POINT ( 'NONE',  ( 34.22339607592780197, -292.9501780530105179, -285.6211290345370344 ) ) ;
#79417=CARTESIAN_POINT ( 'NONE',  ( -1.855147741623635715, -287.9431019466036332, -338.5814770159034879 ) ) ;
#79418=CARTESIAN_POINT ( 'NONE',  ( -92.25824581259320212, -283.4936551033919727, -220.6658124200015152 ) ) ;
#79419=CARTESIAN_POINT ( 'NONE',  ( -106.1091574582985544, -283.4738900177623009, -244.1616575211198210 ) ) ;
#79420=CARTESIAN_POINT ( 'NONE',  ( -45.66936229887300414, -284.3649897682299184, -343.3355026143385658 ) ) ;
#79421=CARTESIAN_POINT ( 'NONE',  ( -62.85223850573094495, -271.7198730222474410, -199.8330166344707379 ) ) ;
#79422=CARTESIAN_POINT ( 'NONE',  ( -109.9297475123722876, -282.6570294379390020, -293.5864144319137381 ) ) ;
#79423=CARTESIAN_POINT ( 'NONE',  ( -111.6669986347971104, -298.4185626549921722, -280.7779907369480270 ) ) ;
#79424=CARTESIAN_POINT ( 'NONE',  ( -59.93403078015445828, -283.7600525545510095, -198.6157637118226376 ) ) ;
#79425=CARTESIAN_POINT ( 'NONE',  ( -100.7806809583330647, -278.9920702566289492, -307.0539792679182938 ) ) ;
#79428=CARTESIAN_POINT ( 'NONE',  ( 22.05517302192838969, -296.1089529876000483, -317.0865489651146163 ) ) ;
#79430=CARTESIAN_POINT ( 'NONE',  ( -92.45437388432198134, -275.8402696378829546, -321.3050878038019960 ) ) ;
#79431=CARTESIAN_POINT ( 'NONE',  ( -113.6544393155528638, -289.6313493334585019, -279.7743230404922770 ) ) ;
#79432=CARTESIAN_POINT ( 'NONE',  ( -67.64210029969706284, -293.8563418431681384, -337.6678152533099819 ) ) ;
#79433=CARTESIAN_POINT ( 'NONE',  ( 5.222301536452737203, -279.3264045942776193, -210.4482709534483718 ) ) ;
#79434=CARTESIAN_POINT ( 'NONE',  ( 53.58861941461584877, -297.3417089811084111, -196.1551220140682119 ) ) ;
#79435=CARTESIAN_POINT ( 'NONE',  ( -37.56817119584607667, -293.3644705745486476, -196.8557868307845808 ) ) ;
#79437=CARTESIAN_POINT ( 'NONE',  ( -90.24546155566609684, -294.2636173749046407, -325.4238810970804252 ) ) ;
#79438=CARTESIAN_POINT ( 'NONE',  ( -61.49784179577256538, -290.9713933351055744, -340.0957667172688161 ) ) ;
#79439=CARTESIAN_POINT ( 'NONE',  ( -41.96955562042941068, -290.2344377489041563, -194.5155052682038672 ) ) ;
#79440=CARTESIAN_POINT ( 'NONE',  ( -53.52055227643713664, -290.6890838165340938, -342.1498333811127281 ) ) ;
#79442=CARTESIAN_POINT ( 'NONE',  ( -8.144672649333537962, -289.4626710412791795, -337.4983290247773198 ) ) ;
#79444=CARTESIAN_POINT ( 'NONE',  ( -1.970357320849683846, -289.7992907308917552, -338.3087215288892367 ) ) ;
#79445=CARTESIAN_POINT ( 'NONE',  ( -103.3406084486018273, -277.0536025502447046, -233.9942250622320046 ) ) ;
#79446=CARTESIAN_POINT ( 'NONE',  ( -97.68296764298989387, -279.5252143768838664, -222.5628363568824284 ) ) ;
#79447=CARTESIAN_POINT ( 'NONE',  ( 15.73588368284072025, -281.9917530765306424, -326.1151706447361676 ) ) ;
#79448=CARTESIAN_POINT ( 'NONE',  ( 34.96402272740579065, -285.2957740353498934, -250.4391930447644654 ) ) ;
#79449=CYLINDRICAL_SURFACE ( 'NONE', #58022, 6.154241149514405151 ) ;
#79450=CARTESIAN_POINT ( 'NONE',  ( 26.61131017849629643, -280.2020895726905678, -308.1571762069452234 ) ) ;
#79451=CARTESIAN_POINT ( 'NONE',  ( -97.71862719584134993, -283.1599014484700660, -225.7826997122473358 ) ) ;
#79453=CARTESIAN_POINT ( 'NONE',  ( -111.0561816299742048, -277.2817698509196589, -250.5906054077842668 ) ) ;
#79455=CARTESIAN_POINT ( 'NONE',  ( -112.8351764029676048, -283.2993139312862354, -284.1521504859274501 ) ) ;
#79456=CARTESIAN_POINT ( 'NONE',  ( -92.14588786008734189, -274.0459058516042887, -221.8935748811241240 ) ) ;
#79458=CARTESIAN_POINT ( 'NONE',  ( -105.4491481205933212, -292.5309694333656125, -241.8059414365591238 ) ) ;
#79459=CARTESIAN_POINT ( 'NONE',  ( -38.36784355044866857, -275.4647907885492373, -193.9572350653712647 ) ) ;
#79460=CARTESIAN_POINT ( 'NONE',  ( 33.26155244526208321, -275.4648697051891872, -288.9962518138122505 ) ) ;
#79461=CARTESIAN_POINT ( 'NONE',  ( -81.30715076739113556, -297.6500928128484702, -331.1232755813418862 ) ) ;
#79462=CARTESIAN_POINT ( 'NONE',  ( -14.95021994006125610, -288.9367112076967601, -344.0892635359948599 ) ) ;
#79463=CARTESIAN_POINT ( 'NONE',  ( 37.44249742371568601, -279.7696412526656218, -281.1610251400859397 ) ) ;
#79464=CARTESIAN_POINT ( 'NONE',  ( 23.97651662818807949, -292.7646071751225918, -223.7660767972780320 ) ) ;
#79465=CARTESIAN_POINT ( 'NONE',  ( -72.73016753408175816, -290.6303589779037111, -206.1865495274964246 ) ) ;
#79466=CARTESIAN_POINT ( 'NONE',  ( -39.08749757054280138, -293.0739058145688887, -345.3408008541252343 ) ) ;
#79469=CARTESIAN_POINT ( 'NONE',  ( -67.82115183211701037, -291.1486429749041918, -203.9471358221020409 ) ) ;
#79471=CARTESIAN_POINT ( 'NONE',  ( 2.608298161699547535, -287.5153819974877933, -204.8110009010750332 ) ) ;
#79472=CARTESIAN_POINT ( 'NONE',  ( 90.32002540683689062, -302.2645883696979467, -200.3030568020284647 ) ) ;
#79473=CARTESIAN_POINT ( 'NONE',  ( -30.62351921889639073, -294.0279162252280685, -346.8312837867644589 ) ) ;
#79474=CARTESIAN_POINT ( 'NONE',  ( -89.56195626523414433, -286.6499411597344533, -214.3753366125651496 ) ) ;
#79475=CARTESIAN_POINT ( 'NONE',  ( -100.9902799089257144, -284.8758363197011363, -234.5103852853930562 ) ) ;
#79476=CARTESIAN_POINT ( 'NONE',  ( 35.52432281150923643, -276.9272797100709909, -259.2649807279888137 ) ) ;
#79477=CARTESIAN_POINT ( 'NONE',  ( 17.34743313830938760, -292.2864250787960145, -321.1641248401943471 ) ) ;
#79478=CARTESIAN_POINT ( 'NONE',  ( -31.50032385928852463, -296.7376799605291353, -344.1943929307040548 ) ) ;
#79479=CARTESIAN_POINT ( 'NONE',  ( 13.99816718743864286, -275.1072423954169608, -322.8851838525761195 ) ) ;
#79482=CARTESIAN_POINT ( 'NONE',  ( -5.810244013500115656, -294.3155083128707474, -340.5858398895014147 ) ) ;
#79483=CARTESIAN_POINT ( 'NONE',  ( 36.41967353032591603, -289.3377154872188157, -259.9568605048786480 ) ) ;
#79484=CARTESIAN_POINT ( 'NONE',  ( -11.03739043055442082, -296.3812685058572356, -195.3700774844024579 ) ) ;
#79485=CARTESIAN_POINT ( 'NONE',  ( 30.43485240474585041, -299.9617133597211023, -193.6581076686333063 ) ) ;
#79486=CARTESIAN_POINT ( 'NONE',  ( -60.01811337110007116, -286.4017656522879065, -200.8652695422702266 ) ) ;
#79488=CARTESIAN_POINT ( 'NONE',  ( -97.50499473779819937, -278.2508875643740112, -222.6830496920694600 ) ) ;
#79489=CARTESIAN_POINT ( 'NONE',  ( -33.43171266986855272, -295.6555849904203228, -347.1728187782676969 ) ) ;
#79490=CARTESIAN_POINT ( 'NONE',  ( -40.31440192102420639, -287.2287054857509929, -346.0804525038054180 ) ) ;
#79491=CARTESIAN_POINT ( 'NONE',  ( -113.5814117173243858, -297.0197540410792385, -259.6237987697339804 ) ) ;
#79492=CARTESIAN_POINT ( 'NONE',  ( 4.512289767942923469, -292.9673261411324461, -210.4632696967629784 ) ) ;
#79495=CARTESIAN_POINT ( 'NONE',  ( 38.91249631477773363, -289.1228280746155406, -274.3670598194632362 ) ) ;
#79496=CARTESIAN_POINT ( 'NONE',  ( -72.02372285203398405, -289.1237833571631768, -198.2697987213421698 ) ) ;
#79498=CARTESIAN_POINT ( 'NONE',  ( -79.84752079386599632, -278.8425664068086007, -206.2147377848810947 ) ) ;
#79499=CARTESIAN_POINT ( 'NONE',  ( -97.37770050020036194, -285.9409996979936750, -315.0344555408725000 ) ) ;
#79500=CARTESIAN_POINT ( 'NONE',  ( -107.3787279982790608, -283.5208898756325766, -239.6769524679706365 ) ) ;
#79501=CARTESIAN_POINT ( 'NONE',  ( -0.2956276393937394831, -286.6357093279124229, -334.9874812043945553 ) ) ;
#79502=CARTESIAN_POINT ( 'NONE',  ( 36.39530495606224036, -277.6345195464417657, -287.8285537934423814 ) ) ;
#79503=CARTESIAN_POINT ( 'NONE',  ( -41.87842166316425363, -298.4857907140830093, -197.4405680706571786 ) ) ;
#79505=CARTESIAN_POINT ( 'NONE',  ( 19.20185852387434622, -292.8984066857074140, -317.3086360680122766 ) ) ;
#79506=CARTESIAN_POINT ( 'NONE',  ( -107.6183121957091231, -278.8138106119273516, -250.5613630033358561 ) ) ;
#79507=CARTESIAN_POINT ( 'NONE',  ( -103.4585046167218394, -278.3229335873307946, -239.0578632570020545 ) ) ;
#79508=CARTESIAN_POINT ( 'NONE',  ( -49.68310194708145389, -274.9780957396689587, -194.6161652946820197 ) ) ;
#79509=CARTESIAN_POINT ( 'NONE',  ( -42.38849121500016537, -278.7847612117595872, -193.9246174181442939 ) ) ;
#79510=CARTESIAN_POINT ( 'NONE',  ( -57.17162103437372878, -168.6543081016745020, -361.5809719840890466 ) ) ;
#79511=CARTESIAN_POINT ( 'NONE',  ( -104.7424857350691951, -298.4474415156828400, -234.2524315420578205 ) ) ;
#79514=CARTESIAN_POINT ( 'NONE',  ( 82.68073018288104947, -297.0543924324409204, -195.4120394483015559 ) ) ;
#79515=CARTESIAN_POINT ( 'NONE',  ( -19.75495865843054943, -287.3633154671680359, -199.1927781317019708 ) ) ;
#79516=CARTESIAN_POINT ( 'NONE',  ( -89.21112516047233498, -287.0948367177936689, -214.7599300756371576 ) ) ;
#79517=CARTESIAN_POINT ( 'NONE',  ( 21.25021873354771174, -287.5134888657170791, -314.0956793298481671 ) ) ;
#79518=CARTESIAN_POINT ( 'NONE',  ( 0.8323737669285214968, -282.0648062477305302, -337.1765393366437138 ) ) ;
#79519=CARTESIAN_POINT ( 'NONE',  ( -101.2860737566626881, -276.4510990783794000, -307.3088494285454999 ) ) ;
#79520=CARTESIAN_POINT ( 'NONE',  ( -111.5525416636177596, -286.3690393845018889, -273.7172119853556183 ) ) ;
#79521=CARTESIAN_POINT ( 'NONE',  ( -83.86055731133599522, -277.8801077595737183, -213.1400002179955777 ) ) ;
#79522=CARTESIAN_POINT ( 'NONE',  ( -102.2849350589290225, -279.4018251965210879, -304.7648926796004503 ) ) ;
#79523=CARTESIAN_POINT ( 'NONE',  ( 13.53501927138226613, -275.2807254340241911, -217.9249866920037562 ) ) ;
#79524=CARTESIAN_POINT ( 'NONE',  ( -3.251298052482054057, -287.4069614254707972, -338.9748915458093279 ) ) ;
#79525=CARTESIAN_POINT ( 'NONE',  ( -88.20697334313787508, -284.5456590274911264, -328.0245384175451022 ) ) ;
#79526=CARTESIAN_POINT ( 'NONE',  ( 37.13381725701844260, -282.2863879334347530, -289.6723637645936265 ) ) ;
#79530=CARTESIAN_POINT ( 'NONE',  ( -82.10351036824796722, -291.5158110587657347, -331.4895550801701916 ) ) ;
#79531=CARTESIAN_POINT ( 'NONE',  ( -108.3470402139863893, -288.8731267976909862, -298.8486582580608797 ) ) ;
#79532=CARTESIAN_POINT ( 'NONE',  ( -89.40103400258027477, -272.3551393946534631, -218.8515634852495282 ) ) ;
#79533=CARTESIAN_POINT ( 'NONE',  ( -2.021693309433206132, -293.9454070276229345, -338.6678519497706361 ) ) ;
#79534=CARTESIAN_POINT ( 'NONE',  ( -69.07390035720762000, -287.9571776946671093, -336.8725848386332018 ) ) ;
#79535=CARTESIAN_POINT ( 'NONE',  ( 35.21425320698516970, -291.6018483156392449, -255.7457954937454190 ) ) ;
#79536=CARTESIAN_POINT ( 'NONE',  ( 18.13568770314636680, -289.4390346597742223, -318.4933462508482194 ) ) ;
#79537=CARTESIAN_POINT ( 'NONE',  ( 21.31550574532285580, -296.6948066931273615, -317.0979686699210447 ) ) ;
#79538=CARTESIAN_POINT ( 'NONE',  ( 20.86940451829296350, -290.2038471250402836, -317.6726484382376157 ) ) ;
#79539=CARTESIAN_POINT ( 'NONE',  ( -80.84802470311109346, -289.4629772922522193, -209.0648852606259425 ) ) ;
#79540=CARTESIAN_POINT ( 'NONE',  ( -110.1219492398727624, -292.7855442334407030, -252.1975282590965719 ) ) ;
#79541=CARTESIAN_POINT ( 'NONE',  ( -97.55621111271682366, -286.0725461758831329, -228.6541632731328377 ) ) ;
#79542=CARTESIAN_POINT ( 'NONE',  ( -41.96721188365903998, -293.9941322660226888, -195.3369014338937575 ) ) ;
#79543=CARTESIAN_POINT ( 'NONE',  ( 121.3887860922853150, -299.5541904835127980, -197.6024395396064222 ) ) ;
#79544=CARTESIAN_POINT ( 'NONE',  ( -112.5415345926156050, -274.6034480829973745, -264.7738583930552636 ) ) ;
#79545=CARTESIAN_POINT ( 'NONE',  ( 20.30189504774060794, -281.3829770374169357, -315.4146157683587148 ) ) ;
#79546=CARTESIAN_POINT ( 'NONE',  ( -2.720183057619603773, -280.5943139236004527, -336.9063337629759758 ) ) ;
#79547=CARTESIAN_POINT ( 'NONE',  ( -95.46606251925892650, -295.0690040304389186, -320.6176331570524098 ) ) ;
#79548=CARTESIAN_POINT ( 'NONE',  ( 35.37319440412365879, -273.6124190639771996, -256.5582875287274192 ) ) ;
#79549=CARTESIAN_POINT ( 'NONE',  ( -88.09483948869231540, -275.8489468249696870, -324.8169077653797672 ) ) ;
#79550=CARTESIAN_POINT ( 'NONE',  ( -109.8467178981870518, -297.7099477150993607, -282.3721910716241723 ) ) ;
#79551=CARTESIAN_POINT ( 'NONE',  ( 32.10208298100891255, -295.3006056983235226, -294.8640815932949408 ) ) ;
#79553=CARTESIAN_POINT ( 'NONE',  ( 18.96390443441587337, -295.0160705867976958, -317.0760044998428953 ) ) ;
#79555=CARTESIAN_POINT ( 'NONE',  ( -24.05069231370500660, -284.2410579614560788, -196.1342339643691162 ) ) ;
#79556=CARTESIAN_POINT ( 'NONE',  ( -77.51197591391908759, -297.4968279394936985, -209.3467125891144747 ) ) ;
#79557=CARTESIAN_POINT ( 'NONE',  ( -113.8196391722676992, -284.6640998759768308, -261.4098700498012136 ) ) ;
#79558=CARTESIAN_POINT ( 'NONE',  ( 23.26818510146473429, -287.8535928152922452, -317.8395440983318281 ) ) ;
#79559=CARTESIAN_POINT ( 'NONE',  ( 24.87940633120200218, -290.9887891372476361, -228.7851352809141190 ) ) ;
#79560=CARTESIAN_POINT ( 'NONE',  ( -97.56395413642863446, -278.3892845631813202, -222.6385976849548456 ) ) ;
#79561=CARTESIAN_POINT ( 'NONE',  ( -69.85430415644619018, -277.1237833571632905, -202.7746430608542312 ) ) ;
#79563=CARTESIAN_POINT ( 'NONE',  ( 35.35151333689758957, -286.4813149617853583, -280.5928645412478772 ) ) ;
#79564=CARTESIAN_POINT ( 'NONE',  ( -89.29222824684700299, -288.6836798894306071, -326.7759665353119658 ) ) ;
#79567=CARTESIAN_POINT ( 'NONE',  ( -111.1842766871718311, -298.1374858967251384, -271.4955286000169963 ) ) ;
#79568=CARTESIAN_POINT ( 'NONE',  ( 1.062004353205869611, -281.9791353082589467, -204.2421091608420625 ) ) ;
#79569=CARTESIAN_POINT ( 'NONE',  ( -92.50301739849227545, -293.8570454071830227, -321.7185741260280452 ) ) ;
#79570=CARTESIAN_POINT ( 'NONE',  ( 20.19500995666101772, -281.8524524261554802, -315.3234853523587162 ) ) ;
#79571=CARTESIAN_POINT ( 'NONE',  ( -1.965589941400027074, -294.7633679942503591, -338.7535944151754279 ) ) ;
#79572=CARTESIAN_POINT ( 'NONE',  ( 20.99431466043375494, -284.9745315258292635, -222.3379612728367078 ) ) ;
#79573=CARTESIAN_POINT ( 'NONE',  ( -45.09268746682259632, -281.9542883499210006, -195.7110931146172277 ) ) ;
#79574=CARTESIAN_POINT ( 'NONE',  ( -95.46853083156980802, -296.2358674631373674, -225.7909410050751546 ) ) ;
#79576=CARTESIAN_POINT ( 'NONE',  ( -56.72219377252064021, -285.2831572637023783, -342.4460905212382613 ) ) ;
#79577=LINE ( 'NONE', #92832, #23200 ) ;
#79578=CARTESIAN_POINT ( 'NONE',  ( -20.25526795762938548, -292.3380690714490129, -345.3683826091709648 ) ) ;
#79579=CARTESIAN_POINT ( 'NONE',  ( 14.76615024828351785, -275.5377154271676545, -326.9041442237817137 ) ) ;
#79582=CARTESIAN_POINT ( 'NONE',  ( -22.73855337868598170, -292.0776122451333094, -198.8366598615854741 ) ) ;
#79583=CARTESIAN_POINT ( 'NONE',  ( 19.90275384531025438, -283.7229086799844708, -316.7898524526663664 ) ) ;
#79585=CARTESIAN_POINT ( 'NONE',  ( -91.72570709149921697, -274.8606373358587120, -220.4543281199715068 ) ) ;
#79586=CARTESIAN_POINT ( 'NONE',  ( -31.67523405404176629, -284.5819051385494163, -346.3632708633675179 ) ) ;
#79587=CARTESIAN_POINT ( 'NONE',  ( 31.72304525629968808, -280.6779260165739629, -295.3546399174426824 ) ) ;
#79588=CARTESIAN_POINT ( 'NONE',  ( -94.22740690673346364, -279.8749314897559657, -319.2386896866080974 ) ) ;
#79589=CARTESIAN_POINT ( 'NONE',  ( -96.02906609762931112, -273.3909868535999408, -220.4931173927418513 ) ) ;
#79590=CARTESIAN_POINT ( 'NONE',  ( 36.49285885468430735, -275.6601306437435142, -292.2584432589188168 ) ) ;
#79591=CARTESIAN_POINT ( 'NONE',  ( 37.05982424243434536, -295.4413531459576348, -267.9679263101124889 ) ) ;
#79594=CARTESIAN_POINT ( 'NONE',  ( -55.79277367233232354, -293.4268250844205568, -343.8448805623857538 ) ) ;
#79595=CARTESIAN_POINT ( 'NONE',  ( -83.22436863694792919, -272.9113761493084098, -213.5036719270056267 ) ) ;
#79596=CARTESIAN_POINT ( 'NONE',  ( 19.84612272703604319, -294.3817145478230941, -219.8214794834491670 ) ) ;
#79597=CARTESIAN_POINT ( 'NONE',  ( -20.19161114001083490, -279.3376638359844719, -345.3538533559490702 ) ) ;
#79598=CARTESIAN_POINT ( 'NONE',  ( 20.99802122446750730, -294.0842113561472502, -220.6974977267844338 ) ) ;
#79599=CARTESIAN_POINT ( 'NONE',  ( 24.27352756056665939, -290.1295099026854132, -312.8524350575557378 ) ) ;
#79600=CARTESIAN_POINT ( 'NONE',  ( -97.58364759989588322, -275.9448053341776586, -314.7778331508105794 ) ) ;
#79601=CARTESIAN_POINT ( 'NONE',  ( -40.54370668040117209, -279.0128535269700478, -344.7449340695518458 ) ) ;
#79602=CARTESIAN_POINT ( 'NONE',  ( 35.63289677954256973, -291.4418613509101306, -255.6634172456244016 ) ) ;
#79603=CARTESIAN_POINT ( 'NONE',  ( 36.93930066030053183, -283.6022140628785451, -285.2821905059549863 ) ) ;
#79605=CARTESIAN_POINT ( 'NONE',  ( 13.93650831662567136, -281.9753456912669094, -322.4191590847545399 ) ) ;
#79606=CARTESIAN_POINT ( 'NONE',  ( -22.63896580860269836, -281.3156362531685772, -195.0387478172308136 ) ) ;
#79607=CARTESIAN_POINT ( 'NONE',  ( -94.11523753974346107, -282.6446987398844612, -321.8079452693061739 ) ) ;
#79608=CARTESIAN_POINT ( 'NONE',  ( -67.28177619227146522, -280.6102570590668392, -199.6758149938056590 ) ) ;
#79610=CARTESIAN_POINT ( 'NONE',  ( 37.26339210323240536, -276.8692583411929604, -254.2748135917506431 ) ) ;
#79611=CARTESIAN_POINT ( 'NONE',  ( -37.37352853689063181, -294.5519495502701375, -200.3611179825600459 ) ) ;
#79613=CARTESIAN_POINT ( 'NONE',  ( -96.06687529340298681, -275.1907627728191983, -223.9781228983767676 ) ) ;
#79614=CARTESIAN_POINT ( 'NONE',  ( -109.7741328044625675, -276.3388494539403268, -288.4524396009228440 ) ) ;
#79615=CARTESIAN_POINT ( 'NONE',  ( -96.68640816631436508, -292.9564122111787583, -222.9039831579609086 ) ) ;
#79616=CARTESIAN_POINT ( 'NONE',  ( 24.93905780996364285, -292.3727207543104214, -231.9896871885923417 ) ) ;
#79617=CARTESIAN_POINT ( 'NONE',  ( -78.10912060702612791, -289.0919170742120627, -335.6731290785575084 ) ) ;
#79619=CARTESIAN_POINT ( 'NONE',  ( 38.02209382081370848, -292.2867499065621928, -283.0460330747451962 ) ) ;
#79620=CARTESIAN_POINT ( 'NONE',  ( -86.24114712889522139, -283.7605477729562153, -215.0182048886497057 ) ) ;
#79621=CARTESIAN_POINT ( 'NONE',  ( -92.60832229505459168, -293.1102152680060158, -220.7793498180965912 ) ) ;
#79622=CARTESIAN_POINT ( 'NONE',  ( -42.70545745607833510, -284.4631602039098652, -196.8504959044786062 ) ) ;
#79623=CARTESIAN_POINT ( 'NONE',  ( -40.23713293684328818, -284.4044841459769941, -343.7972122950033054 ) ) ;
#79625=CARTESIAN_POINT ( 'NONE',  ( -89.32332170511958225, -290.7042778291437344, -326.8476759466742010 ) ) ;
#79626=CARTESIAN_POINT ( 'NONE',  ( 33.51372565921600000, -281.8089371671240428, -252.4918588979496121 ) ) ;
#79627=CARTESIAN_POINT ( 'NONE',  ( 0.3317800932513300660, -293.3568510374392417, -337.0749254412979212 ) ) ;
#79628=CARTESIAN_POINT ( 'NONE',  ( 28.77002472021120383, -288.8662186069650488, -309.5197525057987491 ) ) ;
#79629=CARTESIAN_POINT ( 'NONE',  ( 37.44608017412164003, -288.2712568113029192, -288.4809795075651664 ) ) ;
#79630=CARTESIAN_POINT ( 'NONE',  ( -25.14390984947545249, -286.3785701115285178, -198.3361171684697695 ) ) ;
#79632=CARTESIAN_POINT ( 'NONE',  ( 37.14728970841045452, -295.5894356295896159, -284.2767623477607799 ) ) ;
#79633=CARTESIAN_POINT ( 'NONE',  ( -65.43808186185871989, -294.0966975383515205, -341.5362761815433714 ) ) ;
#79634=CARTESIAN_POINT ( 'NONE',  ( -108.9974715653428206, -277.4119744527378089, -285.4892001009048954 ) ) ;
#79635=CARTESIAN_POINT ( 'NONE',  ( -113.4824750946428367, -272.2026622434643741, -258.9476367018966130 ) ) ;
#79636=CARTESIAN_POINT ( 'NONE',  ( -73.66080764165454298, -294.0235084408667490, -334.4831125120363708 ) ) ;
#79637=CARTESIAN_POINT ( 'NONE',  ( 12.44570241331270211, -278.1078145747293320, -325.1955301150332502 ) ) ;
#79638=CARTESIAN_POINT ( 'NONE',  ( -107.4655436004293705, -271.0103491353746108, -245.9990151154011926 ) ) ;
#79639=CARTESIAN_POINT ( 'NONE',  ( 4.718694414574347462, -293.8389803564352860, -210.1485648752665725 ) ) ;
#79640=CARTESIAN_POINT ( 'NONE',  ( -108.2651507527501451, -297.3873591156042266, -288.9603827133764753 ) ) ;
#79642=CARTESIAN_POINT ( 'NONE',  ( -84.05664340632368692, -295.4115979760393316, -211.4735768728311029 ) ) ;
#79643=CARTESIAN_POINT ( 'NONE',  ( -62.81910683683614138, -298.3804075915904832, -197.8062109545585656 ) ) ;
#79644=CARTESIAN_POINT ( 'NONE',  ( -67.89496029504422836, -275.6512994793333746, -201.8525297004382253 ) ) ;
#79645=CARTESIAN_POINT ( 'NONE',  ( -61.32077575071903652, -290.3126231363195302, -339.5594733111145160 ) ) ;
#79646=CARTESIAN_POINT ( 'NONE',  ( -67.30000412886899142, -295.7894387049378224, -336.9675262229276314 ) ) ;
#79647=CARTESIAN_POINT ( 'NONE',  ( -112.1305238194655658, -280.4089327076480913, -279.9947798280949200 ) ) ;
#79648=CARTESIAN_POINT ( 'NONE',  ( -45.20591423952502197, -278.6394883062625354, -194.2068746254713290 ) ) ;
#79650=CARTESIAN_POINT ( 'NONE',  ( 4.483289176046659996, -281.8527107205018751, -334.9529805667808091 ) ) ;
#79651=CARTESIAN_POINT ( 'NONE',  ( 25.24876753940065655, -274.3079567936619014, -225.6648140162351126 ) ) ;
#79652=CARTESIAN_POINT ( 'NONE',  ( -109.8331002845297917, -282.4124491934122148, -287.3376217508055106 ) ) ;
#79653=CARTESIAN_POINT ( 'NONE',  ( -73.36922729722932957, -277.9823837530858555, -203.2012746820324196 ) ) ;
#79654=CARTESIAN_POINT ( 'NONE',  ( 15.94192959134534782, -278.8044777035839843, -217.2703431897868711 ) ) ;
#79655=CARTESIAN_POINT ( 'NONE',  ( -88.45678501247394365, -296.0024583026014398, -217.4839132598680465 ) ) ;
#79656=CARTESIAN_POINT ( 'NONE',  ( 33.83537121001608483, -277.8596818949843055, -294.1609525081875063 ) ) ;
#79658=CARTESIAN_POINT ( 'NONE',  ( -1.562116348872140792, -290.5441865549014437, -204.0419790453083237 ) ) ;
#79659=CARTESIAN_POINT ( 'NONE',  ( -71.90646914995376449, -289.4964572090494244, -339.1671986910600367 ) ) ;
#79660=CARTESIAN_POINT ( 'NONE',  ( 32.01191956623917179, -277.1731482208267607, -241.2422513616602373 ) ) ;
#79662=CARTESIAN_POINT ( 'NONE',  ( -85.22895706849492115, -295.3892637488935975, -212.7883595114597597 ) ) ;
#79663=CARTESIAN_POINT ( 'NONE',  ( -113.7443915820733196, -283.6469002057568787, -278.5334835406822549 ) ) ;
#79665=CARTESIAN_POINT ( 'NONE',  ( -98.71588300517325365, -283.1375780708503953, -227.2320419190264715 ) ) ;
#79667=CARTESIAN_POINT ( 'NONE',  ( 20.50527407133458269, -291.7135437508745781, -225.1649086648845639 ) ) ;
#79668=CARTESIAN_POINT ( 'NONE',  ( -68.03717204446434152, -283.7843552954169013, -202.7693027462782425 ) ) ;
#79671=CARTESIAN_POINT ( 'NONE',  ( 27.98889783105205353, -291.0600120228335754, -233.4187056126531843 ) ) ;
#79672=CARTESIAN_POINT ( 'NONE',  ( -100.8529238652530466, -282.4692202936761873, -312.7529145065806233 ) ) ;
#79673=CARTESIAN_POINT ( 'NONE',  ( -99.84187348620854152, -279.6150634911273301, -309.7015187993507652 ) ) ;
#79674=CARTESIAN_POINT ( 'NONE',  ( -111.3416731436633142, -286.0086781676909595, -250.3622879153004703 ) ) ;
#79675=CARTESIAN_POINT ( 'NONE',  ( -109.0564216407767191, -279.7607273861166277, -286.9206501410660621 ) ) ;
#79676=CARTESIAN_POINT ( 'NONE',  ( -108.4490203671141870, -279.5816148581252492, -253.1462774101656521 ) ) ;
#79677=CARTESIAN_POINT ( 'NONE',  ( -108.3234055418421633, -286.2390008515696422, -294.5809062667544254 ) ) ;
#79679=CARTESIAN_POINT ( 'NONE',  ( -39.10996669591111186, -294.9070896768083685, -347.3408116548110343 ) ) ;
#79680=CARTESIAN_POINT ( 'NONE',  ( -70.68500753923009938, -291.4739437208638151, -337.1590468390009505 ) ) ;
#79682=CARTESIAN_POINT ( 'NONE',  ( -2.602324593224680793, -285.1233781216987495, -342.4248175857292154 ) ) ;
#79685=CARTESIAN_POINT ( 'NONE',  ( 37.28295724486097384, -292.1468308549264634, -285.7754272365852444 ) ) ;
#79686=CARTESIAN_POINT ( 'NONE',  ( 30.59348526301799254, -288.6911162329827789, -241.6717684374915507 ) ) ;
#79687=CARTESIAN_POINT ( 'NONE',  ( 36.57909759969555807, -283.3604410048124009, -274.0610740006311516 ) ) ;
#79688=CARTESIAN_POINT ( 'NONE',  ( 26.95885546823513579, -289.5242205595983478, -311.7387908025423258 ) ) ;
#79689=CARTESIAN_POINT ( 'NONE',  ( -20.58797924134459123, -290.1566842959712176, -345.0653617365445029 ) ) ;
#79690=CARTESIAN_POINT ( 'NONE',  ( -110.8952605595844858, -286.7405253282360036, -255.7025232408682314 ) ) ;
#79691=CARTESIAN_POINT ( 'NONE',  ( -104.7946081182136595, -279.1998291917834081, -233.2248121867210102 ) ) ;
#79693=CARTESIAN_POINT ( 'NONE',  ( -3.888736827723339395, -292.6942914037786068, -338.1265609784634876 ) ) ;
#79694=CARTESIAN_POINT ( 'NONE',  ( 33.17379529137194538, -280.9910436776739857, -239.4327344128597872 ) ) ;
#79695=CARTESIAN_POINT ( 'NONE',  ( -34.00852999388171582, -275.9549408356749041, -196.2007818257683027 ) ) ;
#79697=CARTESIAN_POINT ( 'NONE',  ( -114.2704648735229114, -287.0519495502703080, -270.3937649182068981 ) ) ;
#79698=CARTESIAN_POINT ( 'NONE',  ( -78.27654851829649374, -271.7494057031277066, -206.3430564706237647 ) ) ;
#79700=CARTESIAN_POINT ( 'NONE',  ( -32.95305800079159297, -279.6165842382140454, -197.4315062872732369 ) ) ;
#79701=CARTESIAN_POINT ( 'NONE',  ( 3.303890688361111660, -277.7242947534754194, -335.3538718953298599 ) ) ;
#79702=CARTESIAN_POINT ( 'NONE',  ( -94.92363777879110387, -298.6193093539531560, -224.5386848785209395 ) ) ;
#79703=CARTESIAN_POINT ( 'NONE',  ( -44.40952714796666356, -282.1981054541017215, -346.8529550229571896 ) ) ;
#79704=CARTESIAN_POINT ( 'NONE',  ( -89.35752196413908166, -291.5571509469536977, -323.0140219024945054 ) ) ;
#79705=CARTESIAN_POINT ( 'NONE',  ( -101.7417216877868356, -298.6136080055156299, -229.4301397984350785 ) ) ;
#79706=CARTESIAN_POINT ( 'NONE',  ( -37.26944708758045977, -299.2581092072196043, -193.7574132542464440 ) ) ;
#79707=CARTESIAN_POINT ( 'NONE',  ( 34.51761467832923103, -295.8223644798799796, -291.2942432471122629 ) ) ;
#79708=CARTESIAN_POINT ( 'NONE',  ( -40.33250351514033127, -281.0896855109197077, -345.1346662736161193 ) ) ;
#79709=CARTESIAN_POINT ( 'NONE',  ( -113.1132439323231011, -290.0480570382330825, -284.0156331628174371 ) ) ;
#79710=CARTESIAN_POINT ( 'NONE',  ( -63.86818523615091436, -271.7246719120348644, -200.5748896092077018 ) ) ;
#79711=CARTESIAN_POINT ( 'NONE',  ( -21.17378137699595086, -287.8563610831972710, -195.8961005807035747 ) ) ;
#79712=CARTESIAN_POINT ( 'NONE',  ( -97.61084208874066803, -288.8932017728215556, -312.1187333311298744 ) ) ;
#79713=CARTESIAN_POINT ( 'NONE',  ( 175.4127752309341304, 242.4573000288498577, -179.5786504745925924 ) ) ;
#79715=CARTESIAN_POINT ( 'NONE',  ( -97.87028991636330488, -289.7542429649195697, -223.7041719871709233 ) ) ;
#79716=CARTESIAN_POINT ( 'NONE',  ( -21.12877183614458687, -288.5050673808910915, -341.5596323131114787 ) ) ;
#79718=CARTESIAN_POINT ( 'NONE',  ( -67.08192969538106354, -286.7509719706591227, -199.6715766379703325 ) ) ;
#79719=CARTESIAN_POINT ( 'NONE',  ( -53.95461655067646234, -277.6044974271193269, -341.5195211759166227 ) ) ;
#79720=CARTESIAN_POINT ( 'NONE',  ( 13.08560285237687637, -291.6580343960332016, -212.5806747248830675 ) ) ;
#79721=CARTESIAN_POINT ( 'NONE',  ( -31.63556441068186231, -283.6333430740610879, -347.0604349262638948 ) ) ;
#79722=CARTESIAN_POINT ( 'NONE',  ( -1.938475530984976380, -284.1119793342703019, -337.9578593420944230 ) ) ;
#79723=CARTESIAN_POINT ( 'NONE',  ( -66.56429172319867860, -283.7578368697517135, -341.5917613937901365 ) ) ;
#79724=CARTESIAN_POINT ( 'NONE',  ( 26.47526072909369432, -281.4003472818442901, -234.8719225330882807 ) ) ;
#79725=CARTESIAN_POINT ( 'NONE',  ( -90.05876305092316159, -230.6096148880447174, -347.9243686835410472 ) ) ;
#79726=CARTESIAN_POINT ( 'NONE',  ( 178.7692323741149778, 254.2009183757706978, -166.1924330971562824 ) ) ;
#79727=CARTESIAN_POINT ( 'NONE',  ( -48.59893405485766493, -154.6077932284252370, -361.6058154342690614 ) ) ;
#79728=CARTESIAN_POINT ( 'NONE',  ( -89.34979084111495240, -272.4935364899786236, -218.9047264724705997 ) ) ;
#79729=CARTESIAN_POINT ( 'NONE',  ( -58.84014220375144077, -294.8305230767922467, -344.2904846600839619 ) ) ;
#79730=CARTESIAN_POINT ( 'NONE',  ( -97.18990753655256754, -247.1757387921193470, -331.6343048592842706 ) ) ;
#79731=CARTESIAN_POINT ( 'NONE',  ( -71.16958532213601529, -272.2997657850657447, -201.7391648030283022 ) ) ;
#79732=CARTESIAN_POINT ( 'NONE',  ( -109.9928112981043284, -298.6112232705164615, -255.0459997793538207 ) ) ;
#79733=CARTESIAN_POINT ( 'NONE',  ( 18.20921659388077885, -289.5491151505507901, -318.5553062109909774 ) ) ;
#79735=CARTESIAN_POINT ( 'NONE',  ( -69.41864491853944230, -296.4052712470773940, -340.1170989780540594 ) ) ;
#79736=CARTESIAN_POINT ( 'NONE',  ( -25.13770793834681072, -286.7041848474858625, -198.2747092675330975 ) ) ;
#79737=CARTESIAN_POINT ( 'NONE',  ( -15.85074699759223016, -273.2440056286607728, -196.6878516768029499 ) ) ;
#79738=CARTESIAN_POINT ( 'NONE',  ( 38.44870992035536261, -294.5144949775105374, -283.0889303090206113 ) ) ;
#79739=CARTESIAN_POINT ( 'NONE',  ( 6.456049935955877395, -293.1223099108862016, -207.1054147423439531 ) ) ;
#79740=CARTESIAN_POINT ( 'NONE',  ( -32.15940456283966853, -292.2859856728004502, -197.5326764645921003 ) ) ;
#79742=CARTESIAN_POINT ( 'NONE',  ( -101.5093032186467497, -275.0041785203033555, -230.4633372124957020 ) ) ;
#79743=CARTESIAN_POINT ( 'NONE',  ( 22.45806013025439896, -273.7022788889118488, -222.4655018231010501 ) ) ;
#79745=CARTESIAN_POINT ( 'NONE',  ( -102.0486346453794226, -277.5121535851188241, -312.0821310875710424 ) ) ;
#79746=CARTESIAN_POINT ( 'NONE',  ( 24.47460512389315213, -273.3994820393477880, -230.0475368970224679 ) ) ;
#79747=CARTESIAN_POINT ( 'NONE',  ( -35.39584491339906691, -275.1567852680404371, -197.0652755013672675 ) ) ;
#79748=CARTESIAN_POINT ( 'NONE',  ( 32.74504452628131190, -276.7742972642525388, -291.6474169475393410 ) ) ;
#79749=CARTESIAN_POINT ( 'NONE',  ( -15.12129468388211073, -299.9260740170659005, -194.1551783861579565 ) ) ;
#79750=CARTESIAN_POINT ( 'NONE',  ( 37.97816042962453764, -273.6186377233868825, -273.9904382731602936 ) ) ;
#79751=CARTESIAN_POINT ( 'NONE',  ( -39.68400421170134962, -295.7337232914933338, -343.4379640680119223 ) ) ;
#79752=CARTESIAN_POINT ( 'NONE',  ( -23.42505242796522325, -293.4456092923480242, -342.6744807516273568 ) ) ;
#79754=CARTESIAN_POINT ( 'NONE',  ( -95.16040015187419954, -278.3570321874347542, -321.1205981897799688 ) ) ;
#79755=CARTESIAN_POINT ( 'NONE',  ( 34.62529726240596517, -275.5564234584599035, -258.0495930198588894 ) ) ;
#79756=CARTESIAN_POINT ( 'NONE',  ( -97.18412775178586571, -283.8793110427347415, -222.6937063541520843 ) ) ;
#79757=CARTESIAN_POINT ( 'NONE',  ( -109.8173961340521885, -298.2965337850353649, -290.2935517826441583 ) ) ;
#79759=CARTESIAN_POINT ( 'NONE',  ( -33.21935644195431081, -285.3024106417127541, -197.2659417829366362 ) ) ;
#79760=CARTESIAN_POINT ( 'NONE',  ( -110.2885886290011115, -276.6281456993712027, -282.9551644455639803 ) ) ;
#79761=CARTESIAN_POINT ( 'NONE',  ( -69.52536840240330207, -276.0589442887876999, -336.5535117712911415 ) ) ;
#79762=CARTESIAN_POINT ( 'NONE',  ( 13.73331525455091295, -284.3369713028795900, -325.3524440498138119 ) ) ;
#79763=CARTESIAN_POINT ( 'NONE',  ( 3.367019751394966676, -277.6963936503413493, -331.4342759974665569 ) ) ;
#79765=CARTESIAN_POINT ( 'NONE',  ( 9.039699025572616620, -273.0767756364499519, -209.9028164353674129 ) ) ;
#79766=CARTESIAN_POINT ( 'NONE',  ( -58.80364107911314875, -281.7753311520498301, -198.3235339397816119 ) ) ;
#79768=CARTESIAN_POINT ( 'NONE',  ( 21.30328137218328877, -290.1238536654252016, -318.0268497199367630 ) ) ;
#79769=CARTESIAN_POINT ( 'NONE',  ( 37.05764643777325773, -291.4252642714020567, -260.4914267720184853 ) ) ;
#79771=CARTESIAN_POINT ( 'NONE',  ( -33.77254241633748677, -296.8927315211543032, -196.9647934452050322 ) ) ;
#79772=CARTESIAN_POINT ( 'NONE',  ( -111.0182778151683181, -288.5738149002780233, -279.4510783813382773 ) ) ;
#79773=CARTESIAN_POINT ( 'NONE',  ( 193.6056169066500274, 279.7126221763799094, -126.0203154767880989 ) ) ;
#79775=CARTESIAN_POINT ( 'NONE',  ( -96.76248456181804158, -288.3842634174589534, -318.2552941413810572 ) ) ;
#79776=CARTESIAN_POINT ( 'NONE',  ( 19.98623883188853156, -283.8029021379052210, -316.8562824770722841 ) ) ;
#79778=CARTESIAN_POINT ( 'NONE',  ( -101.6488117861491389, -283.3291769756244207, -229.8818714122986933 ) ) ;
#79779=CARTESIAN_POINT ( 'NONE',  ( -51.11048966926350090, -284.6567262805410223, -342.7027715736420532 ) ) ;
#79780=CARTESIAN_POINT ( 'NONE',  ( -107.1368458063448372, -285.0648642145199005, -292.2982865964136181 ) ) ;
#79782=CARTESIAN_POINT ( 'NONE',  ( -15.40641620089360586, -290.7496314182230321, -342.5076401081882409 ) ) ;
#79783=CARTESIAN_POINT ( 'NONE',  ( 20.01727652225171283, -275.1882505973370030, -218.9437967455579326 ) ) ;
#79784=CARTESIAN_POINT ( 'NONE',  ( -91.75774017248153314, -289.3640858728285252, -217.8633471467662446 ) ) ;
#79785=CARTESIAN_POINT ( 'NONE',  ( -41.38444542250103098, -277.1017034222018083, -347.2681250818313856 ) ) ;
#79786=CARTESIAN_POINT ( 'NONE',  ( 27.22781193056925275, -296.0345058290855604, -307.8127523001895156 ) ) ;
#79788=CARTESIAN_POINT ( 'NONE',  ( -110.4683760289727132, -293.2662352645559167, -253.7030783399848985 ) ) ;
#79789=CARTESIAN_POINT ( 'NONE',  ( -2.207541027192220007, -281.2616653458595692, -334.9265235211501590 ) ) ;
#79790=CARTESIAN_POINT ( 'NONE',  ( -94.76549965371945916, -275.8824393019547756, -318.8839378697941243 ) ) ;
#79791=CARTESIAN_POINT ( 'NONE',  ( -85.35681618659506853, -271.8820720181499837, -211.0546564393862639 ) ) ;
#79792=CARTESIAN_POINT ( 'NONE',  ( 23.14132724935378249, -274.3303027134767831, -229.2814322489235792 ) ) ;
#79793=CARTESIAN_POINT ( 'NONE',  ( -52.53140921108406047, -293.3743172515387982, -198.1978309387543788 ) ) ;
#79794=CARTESIAN_POINT ( 'NONE',  ( 21.52271486849027227, -295.1023256204480845, -313.9316251609185429 ) ) ;
#79795=CARTESIAN_POINT ( 'NONE',  ( 36.13254401663373727, -294.7118589412373808, -249.3339273290943936 ) ) ;
#79796=CARTESIAN_POINT ( 'NONE',  ( 27.69559526689053897, -295.3987680965234404, -310.7527222208510125 ) ) ;
#79797=CARTESIAN_POINT ( 'NONE',  ( -55.80535979649476275, -295.1297442824593418, -341.0399364581667214 ) ) ;
#79798=CARTESIAN_POINT ( 'NONE',  ( -111.7712605082640067, -292.4337688317439756, -279.5937335224062394 ) ) ;
#79799=CARTESIAN_POINT ( 'NONE',  ( -88.31994807486660193, -283.9096088846833368, -328.1403525627566182 ) ) ;
#79800=CARTESIAN_POINT ( 'NONE',  ( -85.01238711376386448, -271.5418328090391356, -211.4729945612091058 ) ) ;
#79801=CARTESIAN_POINT ( 'NONE',  ( -15.41142531185276354, -286.1615850034717710, -196.4947296879393548 ) ) ;
#79802=CARTESIAN_POINT ( 'NONE',  ( -57.00981470030789211, -279.2868446704456460, -342.4218210285545183 ) ) ;
#79803=ADVANCED_FACE ( 'NONE', ( #74903, #67794 ), #1521, .F. ) ;
#79804=CARTESIAN_POINT ( 'NONE',  ( -93.54934186181309030, -284.0137589679008556, -223.1612078487472672 ) ) ;
#79805=CARTESIAN_POINT ( 'NONE',  ( -97.44214906301210988, -287.9389745432378618, -315.2481274849307056 ) ) ;
#79806=CARTESIAN_POINT ( 'NONE',  ( -33.94653134347471735, -278.2340269338157555, -194.6724245655335324 ) ) ;
#79807=CARTESIAN_POINT ( 'NONE',  ( 188.7508426036948208, 279.9709457756753181, -124.8390596414617590 ) ) ;
#79808=CARTESIAN_POINT ( 'NONE',  ( -79.33953777290703613, -284.9759729142399465, -210.5146487365948644 ) ) ;
#79809=CARTESIAN_POINT ( 'NONE',  ( 37.28715798272640569, -282.5393574549117375, -253.0251618483688105 ) ) ;
#79810=CARTESIAN_POINT ( 'NONE',  ( -43.17640360332320881, -288.1828827333312120, -346.9037626215624641 ) ) ;
#79811=CARTESIAN_POINT ( 'NONE',  ( -92.73824779070713475, -279.4296111807388456, -322.7594912745115039 ) ) ;
#79812=CARTESIAN_POINT ( 'NONE',  ( -77.54143906954840304, -278.8944476439708637, -335.5170619407300592 ) ) ;
#79813=CARTESIAN_POINT ( 'NONE',  ( -108.6062910400219010, -278.5948870703792863, -254.4811943813358823 ) ) ;
#79814=CARTESIAN_POINT ( 'NONE',  ( -16.19838241306328541, -276.3066017305691844, -198.7194715564970693 ) ) ;
#79815=CARTESIAN_POINT ( 'NONE',  ( 23.10807104604907991, -292.9140081826763549, -222.6449212539245650 ) ) ;
#79816=CARTESIAN_POINT ( 'NONE',  ( -67.00535508885486990, -287.4628433758500137, -338.9139115621897531 ) ) ;
#79817=CARTESIAN_POINT ( 'NONE',  ( -76.77291679176552464, -293.1340749037259457, -205.0958116347061093 ) ) ;
#79818=CARTESIAN_POINT ( 'NONE',  ( -92.97002897682892808, -296.1495177474625962, -222.5954517256548684 ) ) ;
#79819=CARTESIAN_POINT ( 'NONE',  ( 35.55607470134342663, -293.1523756714088336, -265.3191091150566194 ) ) ;
#79820=CARTESIAN_POINT ( 'NONE',  ( -114.0599762162293587, -291.6567426951565949, -268.3764867220202746 ) ) ;
#79821=CARTESIAN_POINT ( 'NONE',  ( 35.24202269008107891, -282.3234664588486567, -279.4627077061001046 ) ) ;
#79822=CARTESIAN_POINT ( 'NONE',  ( -101.0066746986631756, -272.1787837492568656, -227.3760495772780246 ) ) ;
#79823=CARTESIAN_POINT ( 'NONE',  ( -57.25649096048846332, -289.9538607843977616, -344.6907327782436710 ) ) ;
#79824=CARTESIAN_POINT ( 'NONE',  ( -60.87094439978719862, -281.4937416184585004, -342.4345254973252395 ) ) ;
#79825=CARTESIAN_POINT ( 'NONE',  ( -73.16026383770426378, -289.8470415543192757, -338.5137800806448922 ) ) ;
#79827=CARTESIAN_POINT ( 'NONE',  ( -62.57416165117810181, -286.0479747758561757, -201.7841284922041609 ) ) ;
#79828=CARTESIAN_POINT ( 'NONE',  ( 138.5464852711123740, 180.7133914995600605, -241.3450704663493980 ) ) ;
#79829=CARTESIAN_POINT ( 'NONE',  ( 201.2091094121765309, 294.9047486845406070, -68.44675130712812461 ) ) ;
#79830=CARTESIAN_POINT ( 'NONE',  ( -70.05943696497188000, -195.9697670439899468, -356.6292458268069367 ) ) ;
#79831=CARTESIAN_POINT ( 'NONE',  ( -69.80275346352172505, -278.8105541970789432, -204.7813850437195242 ) ) ;
#79832=CARTESIAN_POINT ( 'NONE',  ( 5.113308282586055853, -279.5618692936172920, -210.5965939430733158 ) ) ;
#79833=CARTESIAN_POINT ( 'NONE',  ( -7.694797567457321463, -274.0968230335276985, -199.2636629006667306 ) ) ;
#79834=CARTESIAN_POINT ( 'NONE',  ( -68.71647568833768105, -197.0276430710098055, -358.0455354867054325 ) ) ;
#79835=CARTESIAN_POINT ( 'NONE',  ( -92.63473493410921833, -277.8542020889144624, -217.5476352127069788 ) ) ;
#79836=CARTESIAN_POINT ( 'NONE',  ( -10.40523634634057970, -280.7191817187670040, -340.0310800157167819 ) ) ;
#79837=CARTESIAN_POINT ( 'NONE',  ( 1.274034075506777386, -296.3039225032662216, -335.8042160562505387 ) ) ;
#79838=CARTESIAN_POINT ( 'NONE',  ( -67.83258378651797216, -292.1331780359816435, -203.9523832654658690 ) ) ;
#79839=CARTESIAN_POINT ( 'NONE',  ( -95.35008102488841075, -288.6052747018987361, -315.5065186471342145 ) ) ;
#79840=CARTESIAN_POINT ( 'NONE',  ( 7.169222101908442113, -275.2921030056748464, -207.5893910037138426 ) ) ;
#79841=CARTESIAN_POINT ( 'NONE',  ( -96.40716397846081520, -296.1182186694284155, -313.2808328441833510 ) ) ;
#79845=CARTESIAN_POINT ( 'NONE',  ( -83.70304457559441857, -281.3421346610602427, -210.6296572334624102 ) ) ;
#79846=CARTESIAN_POINT ( 'NONE',  ( -51.90214896488578233, -280.9412415782480252, -198.4605801171763915 ) ) ;
#79847=CARTESIAN_POINT ( 'NONE',  ( -76.98325603881406209, -281.2893712374980737, -205.4733405268882223 ) ) ;
#79848=CARTESIAN_POINT ( 'NONE',  ( -3.523351928541757605, -281.6530512183750261, -335.3345990390674842 ) ) ;
#79849=CIRCLE ( 'NONE', #35991, 2.395975569037533948 ) ;
#79850=CARTESIAN_POINT ( 'NONE',  ( -13.82604475682353673, -272.8428140176880561, -200.5204299557864545 ) ) ;
#79853=CARTESIAN_POINT ( 'NONE',  ( 26.79014666220401963, -275.7972460815495310, -228.0377787043189244 ) ) ;
#79855=CARTESIAN_POINT ( 'NONE',  ( 11.42402705322856704, -278.3760872167123921, -327.3427334237465516 ) ) ;
#79856=CARTESIAN_POINT ( 'NONE',  ( -112.4894782852300352, -276.9516129134252083, -284.2684767926167524 ) ) ;
#79859=CARTESIAN_POINT ( 'NONE',  ( -69.73960393270914437, -285.4563899947398227, -338.4104262511389720 ) ) ;
#79861=CARTESIAN_POINT ( 'NONE',  ( -44.30541898871909012, -291.1591296860802345, -197.4808783274968391 ) ) ;
#79862=CARTESIAN_POINT ( 'NONE',  ( -29.46512029369100816, -285.4980330182161765, -193.8675085985707653 ) ) ;
#79863=CARTESIAN_POINT ( 'NONE',  ( -76.68450266871816723, -281.8260202464169311, -333.1123927796631961 ) ) ;
#79864=CARTESIAN_POINT ( 'NONE',  ( -4.581021098104332445, -281.1864790698703018, -336.2558281527755071 ) ) ;
#79865=CARTESIAN_POINT ( 'NONE',  ( 21.33654561775109570, -283.3732071112323752, -314.4726392767776133 ) ) ;
#79866=CARTESIAN_POINT ( 'NONE',  ( -68.00251869574032071, -271.6494982643052936, -201.9006614263446977 ) ) ;
#79867=CARTESIAN_POINT ( 'NONE',  ( -87.21083404300115660, -283.7709606333540933, -212.6760917204390182 ) ) ;
#79868=CARTESIAN_POINT ( 'NONE',  ( -108.8841400751690855, -298.2614116142880221, -292.9136088955336845 ) ) ;
#79869=CARTESIAN_POINT ( 'NONE',  ( -94.13055417397667668, -280.1458524817245461, -224.1179076155090968 ) ) ;
#79870=CARTESIAN_POINT ( 'NONE',  ( -36.60950086985666729, -288.0614788464633875, -195.1852852343108964 ) ) ;
#79873=CARTESIAN_POINT ( 'NONE',  ( 31.99315808284682561, -295.0822804223934668, -240.3279424557018160 ) ) ;
#79874=CARTESIAN_POINT ( 'NONE',  ( -73.83689859351970597, -275.5365553437517860, -335.8976569923572129 ) ) ;
#79875=CARTESIAN_POINT ( 'NONE',  ( -54.47557780599484545, -288.4639132481751176, -345.3195820339592501 ) ) ;
#79876=CARTESIAN_POINT ( 'NONE',  ( 26.94130282669514287, -291.4599797080752523, -234.0057103104477392 ) ) ;
#79877=CARTESIAN_POINT ( 'NONE',  ( -39.18681828117371424, -275.7606134426038125, -343.8311051767138338 ) ) ;
#79878=CARTESIAN_POINT ( 'NONE',  ( -89.38440831716744128, -293.9336602493576152, -323.3712896321620178 ) ) ;
#79879=CARTESIAN_POINT ( 'NONE',  ( -108.2319702859349917, -292.1217337316521139, -250.9752190893022146 ) ) ;
#79880=CARTESIAN_POINT ( 'NONE',  ( 21.31550574532285580, -284.6948066931273615, -317.0979686699210447 ) ) ;
#79881=CARTESIAN_POINT ( 'NONE',  ( -32.07982067835222040, -293.4668207671824689, -346.4992843907436963 ) ) ;
#79882=CARTESIAN_POINT ( 'NONE',  ( -7.880600594848340634, -290.2598379940407085, -338.0802540273634236 ) ) ;
#79883=CARTESIAN_POINT ( 'NONE',  ( -111.8784507633417320, -288.6039563654632047, -285.2003459329209250 ) ) ;
#79884=CARTESIAN_POINT ( 'NONE',  ( -7.966734408126454170, -290.0850101629147275, -337.8877160459251741 ) ) ;
#79886=CARTESIAN_POINT ( 'NONE',  ( -66.38374255004870861, -290.2451184653572227, -337.5655399012031808 ) ) ;
#79888=DIRECTION ( 'NONE',  ( 0.000000000000000000, 0.000000000000000000, -1.000000000000000000 ) ) ;
#79889=CIRCLE ( 'NONE', #58747, 1.895975569037589015 ) ;
#79890=CARTESIAN_POINT ( 'NONE',  ( -12.33875515447740057, -289.9392085087940814, -342.8243124132956723 ) ) ;
#79891=CARTESIAN_POINT ( 'NONE',  ( -98.89066618633617622, -277.1601291171922981, -226.8854744426099046 ) ) ;
#79892=CARTESIAN_POINT ( 'NONE',  ( -111.7117015696642284, -279.1348734310820419, -250.4394553235269711 ) ) ;
#79893=CARTESIAN_POINT ( 'NONE',  ( -18.92756791313701470, -282.4882215368415928, -345.1600497893560942 ) ) ;
#79894=CARTESIAN_POINT ( 'NONE',  ( 23.57156966168662748, -286.1473971553756428, -314.1169657524922627 ) ) ;
#79896=CARTESIAN_POINT ( 'NONE',  ( 35.78791346908104032, -279.5261541726940777, -257.5969064170384968 ) ) ;
#79897=CARTESIAN_POINT ( 'NONE',  ( -112.3259607959232369, -282.5929181911311616, -267.1733319830004234 ) ) ;
#79899=CARTESIAN_POINT ( 'NONE',  ( -110.6656060873578866, -277.2993212123437274, -249.2350069280225284 ) ) ;
#79900=CARTESIAN_POINT ( 'NONE',  ( -107.9479561542274269, -283.0883590823062832, -300.4344498108670791 ) ) ;
#79901=CARTESIAN_POINT ( 'NONE',  ( -63.37371358197463422, -274.5069477677270129, -201.9740901222407672 ) ) ;
#79902=CARTESIAN_POINT ( 'NONE',  ( -36.21412570704001155, -293.6666153956381891, -196.5571161702578422 ) ) ;
#79903=CARTESIAN_POINT ( 'NONE',  ( -20.66061182921227868, -299.5720516418535908, -193.8506246229822807 ) ) ;
#79904=CARTESIAN_POINT ( 'NONE',  ( 34.72732613703151827, -275.3778995498079780, -282.4199555964726756 ) ) ;
#79905=CARTESIAN_POINT ( 'NONE',  ( -85.75008630428908418, -297.7219809968311210, -327.7147881947425390 ) ) ;
#79906=CARTESIAN_POINT ( 'NONE',  ( -4.331139422035541031, -288.7956889184557667, -339.9406958813351594 ) ) ;
#79907=CARTESIAN_POINT ( 'NONE',  ( 36.28009133020469079, -279.4146336464697811, -253.2998946405561469 ) ) ;
#79908=CARTESIAN_POINT ( 'NONE',  ( -22.19171153026570309, -292.0742309712779274, -194.8119053491355146 ) ) ;
#79910=CARTESIAN_POINT ( 'NONE',  ( -25.35882353113471765, -291.2672470410496430, -198.0611564523699144 ) ) ;
#79911=CARTESIAN_POINT ( 'NONE',  ( -82.98867488528608760, -293.6761491365228949, -329.9358940420221984 ) ) ;
#79914=CARTESIAN_POINT ( 'NONE',  ( -109.6847675829058062, -289.9239003186769423, -280.6719363891194234 ) ) ;
#79916=CARTESIAN_POINT ( 'NONE',  ( -21.04563713393467239, -287.1975907259961218, -195.3460625391977885 ) ) ;
#79917=CARTESIAN_POINT ( 'NONE',  ( -37.30987171927208124, -285.5519495502701375, -340.3611179825599606 ) ) ;
#79918=CARTESIAN_POINT ( 'NONE',  ( -41.94347497937574332, -294.1674237464262660, -347.0400035895781343 ) ) ;
#79919=CARTESIAN_POINT ( 'NONE',  ( 29.34035161715986817, -283.3583025725668563, -307.9764932696696746 ) ) ;
#79920=CARTESIAN_POINT ( 'NONE',  ( -108.9285500315818211, -284.5740352333848477, -256.0669609447368202 ) ) ;
#79921=CARTESIAN_POINT ( 'NONE',  ( 36.07867515015146864, -276.8114173546283041, -266.0937540317375465 ) ) ;
#79922=CARTESIAN_POINT ( 'NONE',  ( -23.23209896148750175, -292.8910786604667464, -343.7130360337502566 ) ) ;
#79923=CARTESIAN_POINT ( 'NONE',  ( -8.597239220105997504, -275.4623156698458502, -337.9090681178068962 ) ) ;
#79926=CARTESIAN_POINT ( 'NONE',  ( -58.84948391120601485, -294.9895634868346406, -344.3298648438227474 ) ) ;
#79927=CARTESIAN_POINT ( 'NONE',  ( 11.06995656023202379, -290.2964621124732503, -326.9768459337045670 ) ) ;
#79928=CARTESIAN_POINT ( 'NONE',  ( -99.67834943728260555, -298.2261617960509170, -225.6885910435495646 ) ) ;
#79930=CARTESIAN_POINT ( 'NONE',  ( 11.19555105210906554, -287.3967987892851284, -215.6302564566073556 ) ) ;
#79931=CARTESIAN_POINT ( 'NONE',  ( -77.70142338315010022, -276.6383853776532646, -335.7215389375089671 ) ) ;
#79932=CARTESIAN_POINT ( 'NONE',  ( 1.724805285077424921, -295.1953733679792435, -336.5964630889572504 ) ) ;
#79933=CARTESIAN_POINT ( 'NONE',  ( -2.391919785929478515, -286.7342947079240503, -337.5832745760851594 ) ) ;
#79934=CARTESIAN_POINT ( 'NONE',  ( -113.3693350731649048, -297.0373969254639519, -258.2134636440722488 ) ) ;
#79935=CARTESIAN_POINT ( 'NONE',  ( -106.5926890010002097, -291.1929369843527411, -247.2010655887430346 ) ) ;
#79938=CARTESIAN_POINT ( 'NONE',  ( -104.9195836729417977, -260.6502345264940459, -315.6181490027205427 ) ) ;
#79939=CARTESIAN_POINT ( 'NONE',  ( 38.40479664784151481, -289.1941171461741646, -280.0160790089450984 ) ) ;
#79940=CARTESIAN_POINT ( 'NONE',  ( -88.47809603358389552, -282.9094976428776249, -206.1857440867352693 ) ) ;
#79942=CARTESIAN_POINT ( 'NONE',  ( -109.5076500699411071, -278.2385931900018932, -243.6482815798421484 ) ) ;
#79943=CARTESIAN_POINT ( 'NONE',  ( -45.82256336789456697, -285.1599463812947306, -344.7646078431207002 ) ) ;
#79944=CARTESIAN_POINT ( 'NONE',  ( -107.6918058678267585, -282.7428138117067533, -300.3205173699818147 ) ) ;
#79945=CARTESIAN_POINT ( 'NONE',  ( -23.54174446356137906, -286.9543820970414458, -343.5635115681350271 ) ) ;
#79946=CARTESIAN_POINT ( 'NONE',  ( 8.740004514686489756, -276.5367630015933855, -210.2214307949028580 ) ) ;
#79947=CARTESIAN_POINT ( 'NONE',  ( -69.29010129422182729, -298.1123846191018743, -204.6550444062928875 ) ) ;
#79948=CARTESIAN_POINT ( 'NONE',  ( -20.75303642919150704, -293.5196797168992475, -342.0100779569017391 ) ) ;
#79949=CARTESIAN_POINT ( 'NONE',  ( -94.89102175147579032, -279.8954836203067202, -219.3573106007924309 ) ) ;
#79950=CARTESIAN_POINT ( 'NONE',  ( 18.30841142094000062, -276.2239205521714211, -317.6058540341190337 ) ) ;
#79951=CARTESIAN_POINT ( 'NONE',  ( -109.2308386884985225, -278.0754224500493592, -257.1004835535222810 ) ) ;
#79952=CARTESIAN_POINT ( 'NONE',  ( 36.28519919539937888, -276.3594897275684161, -248.7147107484173603 ) ) ;
#79953=CARTESIAN_POINT ( 'NONE',  ( -8.015609246350436479, -275.5972297308974817, -341.2376958474231401 ) ) ;
#79955=CARTESIAN_POINT ( 'NONE',  ( -6.903917639956217656, -274.6525737147940731, -338.9208695825799964 ) ) ;
#79956=CARTESIAN_POINT ( 'NONE',  ( -107.2414162518167444, -298.3757202813615663, -239.3654275940185698 ) ) ;
#79961=CARTESIAN_POINT ( 'NONE',  ( -52.16481256535811895, -286.9375687067379204, -198.5662615489234497 ) ) ;
#79962=CARTESIAN_POINT ( 'NONE',  ( -21.22108779242348220, -288.0163481712660882, -196.1041326598771377 ) ) ;
#79963=CARTESIAN_POINT ( 'NONE',  ( 23.62365487127207331, -286.3407795619510239, -229.9319036039915432 ) ) ;
#79964=CARTESIAN_POINT ( 'NONE',  ( -92.79625131606731259, -277.6397508784987735, -221.6465908577899881 ) ) ;
#79965=CARTESIAN_POINT ( 'NONE',  ( -95.09774491985504596, -287.0613183289924564, -223.7029439125718113 ) ) ;
#79966=CARTESIAN_POINT ( 'NONE',  ( -81.68983269541402592, -277.9161220652369479, -211.4417152010780967 ) ) ;
#79967=CARTESIAN_POINT ( 'NONE',  ( 5.699065214431824344, -277.7707387009219815, -329.9952397558817552 ) ) ;
#79968=CARTESIAN_POINT ( 'NONE',  ( 35.08068306358324406, -275.9174022139249587, -260.7181488081261023 ) ) ;
#79969=CARTESIAN_POINT ( 'NONE',  ( 37.43397358022727417, -286.5569129268970414, -287.0524653630985199 ) ) ;
#79970=CARTESIAN_POINT ( 'NONE',  ( 37.03807558136119837, -282.5968231149676058, -289.6434359555658489 ) ) ;
#79971=CARTESIAN_POINT ( 'NONE',  ( 38.08645936024664991, -282.2343665800169106, -285.5308134196599212 ) ) ;
#79972=ORIENTED_EDGE ( 'NONE', *, *, #43878, .T. ) ;
#79975=CARTESIAN_POINT ( 'NONE',  ( 22.32953270403515234, -290.0469348575391564, -317.0687316798927782 ) ) ;
#79976=CARTESIAN_POINT ( 'NONE',  ( -72.95923524778829972, -288.1988528254501034, -338.0861162919775325 ) ) ;
#79977=CARTESIAN_POINT ( 'NONE',  ( -3.564872984653602916, -296.2140040951331343, -338.6805230108923865 ) ) ;
#79979=CARTESIAN_POINT ( 'NONE',  ( -63.37920834285855420, -272.7631445555286405, -201.8971866738182825 ) ) ;
#79980=CARTESIAN_POINT ( 'NONE',  ( -37.78610623516770062, -291.3953133248352287, -193.4643346273714428 ) ) ;
#79981=CARTESIAN_POINT ( 'NONE',  ( 26.98192819670782328, -285.5435407426504639, -234.2958712719755283 ) ) ;
#79982=CARTESIAN_POINT ( 'NONE',  ( 34.91528106421958455, -288.9263050095711947, -283.2475129211538842 ) ) ;
#79983=CARTESIAN_POINT ( 'NONE',  ( -95.95921662488163406, -298.4090924074130271, -317.1477375740089997 ) ) ;
#79984=CARTESIAN_POINT ( 'NONE',  ( 21.72843739972778820, -290.1866567700773771, -316.5956507077469269 ) ) ;
#79985=CARTESIAN_POINT ( 'NONE',  ( -48.61969054578635507, -287.1951287119247809, -344.7295616695670901 ) ) ;
#79986=CARTESIAN_POINT ( 'NONE',  ( -65.06310639938220675, -291.4143486903820417, -340.1041648955310848 ) ) ;
#79987=CARTESIAN_POINT ( 'NONE',  ( -109.4267519983705625, -285.6643402697250735, -257.3617106583516261 ) ) ;
#79988=CARTESIAN_POINT ( 'NONE',  ( -50.27652232133611676, -293.8875607083857062, -196.3157346106499972 ) ) ;
#79991=CARTESIAN_POINT ( 'NONE',  ( -23.70910264812068391, -300.1416918350858509, -194.7966907522588258 ) ) ;
#79992=CARTESIAN_POINT ( 'NONE',  ( 34.38697248441357601, -280.9397964164568293, -284.8324262705728529 ) ) ;
#79993=CARTESIAN_POINT ( 'NONE',  ( -72.36480030478240622, -281.5155043536400399, -336.6814248679848447 ) ) ;
#79994=CARTESIAN_POINT ( 'NONE',  ( -108.2300332706132053, -295.3698936014358196, -300.1468560865658901 ) ) ;
#79995=CARTESIAN_POINT ( 'NONE',  ( 35.11795074634553515, -273.5949247230411743, -255.2136346269770399 ) ) ;
#79996=CARTESIAN_POINT ( 'NONE',  ( -110.5438000832981800, -276.8068866377743689, -256.8419921949972604 ) ) ;
#79997=CARTESIAN_POINT ( 'NONE',  ( -58.05973178621965047, -299.0939771850914894, -199.8486606356547952 ) ) ;
#79999=CARTESIAN_POINT ( 'NONE',  ( -93.91235873392774636, -294.0943731290846586, -321.1124987588493127 ) ) ;
#80000=CARTESIAN_POINT ( 'NONE',  ( 18.43077764739624058, -295.6558161930612414, -318.3887286531371501 ) ) ;
#80002=CARTESIAN_POINT ( 'NONE',  ( -12.94477971193989063, -295.5298057413509696, -339.3883471459948282 ) ) ;
#80004=CARTESIAN_POINT ( 'NONE',  ( -79.98617567928744165, -283.4988497948511394, -208.1704121334990418 ) ) ;
#80005=CARTESIAN_POINT ( 'NONE',  ( -101.2145643573273333, -297.0352209466540216, -235.0162850482779220 ) ) ;
#80006=CARTESIAN_POINT ( 'NONE',  ( -102.5184744938278811, -285.0890344761562005, -229.3612633087130348 ) ) ;
#80007=CARTESIAN_POINT ( 'NONE',  ( 6.117149482042417041, -284.3880909399846360, -332.2364601830437891 ) ) ;
#80008=CARTESIAN_POINT ( 'NONE',  ( 25.83192350677454741, -287.8013541471643748, -314.4394225964033467 ) ) ;
#80009=CARTESIAN_POINT ( 'NONE',  ( -5.232458347296809364, -290.4755195702724109, -202.7524236615331006 ) ) ;
#80010=CARTESIAN_POINT ( 'NONE',  ( -90.93819492506491997, -278.5121184660077915, -215.2272153831272874 ) ) ;
#80011=CARTESIAN_POINT ( 'NONE',  ( 10.64812456238590599, -272.1952119285918457, -210.2361428286349394 ) ) ;
#80013=CARTESIAN_POINT ( 'NONE',  ( 36.05209293348595878, -286.3561750816983817, -271.0551234927905284 ) ) ;
#80014=CARTESIAN_POINT ( 'NONE',  ( -91.39047781611820653, -288.7194067818076064, -324.8437593957765444 ) ) ;
#80017=CARTESIAN_POINT ( 'NONE',  ( -106.7325017251612849, -297.8194117279311968, -295.6380863095468499 ) ) ;
#80018=CARTESIAN_POINT ( 'NONE',  ( -113.7886835724599877, -279.9975413868086775, -268.7648085828665216 ) ) ;
#80019=CARTESIAN_POINT ( 'NONE',  ( -91.53207783417578014, -293.8393373403799842, -322.7234113468590522 ) ) ;
#80020=CARTESIAN_POINT ( 'NONE',  ( -3.135430944350504401, -280.1838368289979826, -205.8332268616105978 ) ) ;
#80021=CARTESIAN_POINT ( 'NONE',  ( -3.226874230951582323, -294.7807877499909068, -339.4059955904979802 ) ) ;
#80022=CARTESIAN_POINT ( 'NONE',  ( 36.32137750142408805, -285.4169195126616501, -253.4790698470454799 ) ) ;
#80023=CARTESIAN_POINT ( 'NONE',  ( -42.32332224370642138, -281.9894799687002660, -195.5267402488123878 ) ) ;
#80024=CIRCLE ( 'NONE', #81485, 2.888540232138026020 ) ;
#80025=CARTESIAN_POINT ( 'NONE',  ( -108.0597480763344578, -295.8620961743175712, -251.2769069749305402 ) ) ;
#80027=CARTESIAN_POINT ( 'NONE',  ( 19.76871431689382419, -284.1999257070568774, -318.4460008600389074 ) ) ;
#80029=CARTESIAN_POINT ( 'NONE',  ( 21.31550574532286291, -284.4094976428775681, -223.6242672951989618 ) ) ;
#80030=CARTESIAN_POINT ( 'NONE',  ( -66.15715898127736239, -272.8816433292671491, -199.1161694326408451 ) ) ;
#80031=CARTESIAN_POINT ( 'NONE',  ( -87.92906026335599279, -291.1543227752288203, -217.6612417906548558 ) ) ;
#80032=CARTESIAN_POINT ( 'NONE',  ( 11.75345746763725430, -282.2689564493453531, -215.4031954281252297 ) ) ;
#80033=CARTESIAN_POINT ( 'NONE',  ( -54.41618812260297489, -275.4292610621345148, -198.5634698823040480 ) ) ;
#80034=CARTESIAN_POINT ( 'NONE',  ( 36.77505886944704372, -283.3765655310703551, -288.1127834550392777 ) ) ;
#80035=CARTESIAN_POINT ( 'NONE',  ( 17.36898165654053727, -279.6509012852746991, -221.4339087422084731 ) ) ;
#80036=CARTESIAN_POINT ( 'NONE',  ( -102.3027338737512508, -280.0508082347383265, -307.9495553102573240 ) ) ;
#80037=CARTESIAN_POINT ( 'NONE',  ( -106.8441332339289715, -273.1437039252710406, -237.2188217909673256 ) ) ;
#80039=CARTESIAN_POINT ( 'NONE',  ( -49.71714681559193139, -273.7319449527918778, -194.3083106230838553 ) ) ;
#80040=CARTESIAN_POINT ( 'NONE',  ( 13.35309030582427248, -296.2569560945738090, -324.9419021120316415 ) ) ;
#80043=FACE_OUTER_BOUND ( 'NONE', #65531, .T. ) ;
#80044=CARTESIAN_POINT ( 'NONE',  ( 34.31040194425124668, -292.0089716057115083, -295.1445308390067908 ) ) ;
#80045=CARTESIAN_POINT ( 'NONE',  ( -91.16362954964095877, -272.7684995182736998, -220.9342165796247741 ) ) ;
#80046=CARTESIAN_POINT ( 'NONE',  ( 18.89151087673606710, -294.3641074791419214, -218.7807560890122431 ) ) ;
#80047=CARTESIAN_POINT ( 'NONE',  ( -4.771743288812468897, -285.1233781216987495, -337.9199732462171255 ) ) ;
#80048=CARTESIAN_POINT ( 'NONE',  ( -68.18305035320545926, -292.8611357790121019, -200.2267849081509894 ) ) ;
#80049=CARTESIAN_POINT ( 'NONE',  ( -67.03358679442662549, -291.4422528928395764, -339.1072389326330949 ) ) ;
#80050=CARTESIAN_POINT ( 'NONE',  ( 22.28260205754713397, -274.1719576849306463, -315.5824737641199818 ) ) ;
#80051=CARTESIAN_POINT ( 'NONE',  ( -13.29759323602683985, -278.6577339457459743, -340.8652588854280339 ) ) ;
#80052=CARTESIAN_POINT ( 'NONE',  ( 34.83643286206906708, -291.8676917096804004, -288.5718653311324715 ) ) ;
#80053=CARTESIAN_POINT ( 'NONE',  ( 37.65207086886465504, -283.5496012573414077, -281.1425739204342449 ) ) ;
#80054=EDGE_LOOP ( 'NONE', ( #91700, #39410, #30471, #12475, #53491 ) ) ;
#80055=CARTESIAN_POINT ( 'NONE',  ( -56.32848531964684469, -282.9703562229142904, -340.8706171637004445 ) ) ;
#80056=CARTESIAN_POINT ( 'NONE',  ( -25.45710659807634002, -281.2799010523970651, -194.5966873725202220 ) ) ;
#80057=CARTESIAN_POINT ( 'NONE',  ( 26.38301014091384999, -280.9095573587291028, -312.8719403645106922 ) ) ;
#80058=CARTESIAN_POINT ( 'NONE',  ( -2.820151828116852055, -277.5483514206277391, -338.9401955847702652 ) ) ;
#80060=CARTESIAN_POINT ( 'NONE',  ( 38.93132166715036391, -277.1180885344637659, -273.9914976001100513 ) ) ;
#80061=CARTESIAN_POINT ( 'NONE',  ( 34.45848030099739390, -290.0519495502701943, -270.3284710469131937 ) ) ;
#80063=CARTESIAN_POINT ( 'NONE',  ( -98.52875165703105154, -299.1417535804828276, -226.9889451591008367 ) ) ;
#80064=CARTESIAN_POINT ( 'NONE',  ( -111.5418660780091784, -276.4613905579420248, -278.9546892281958321 ) ) ;
#80065=CARTESIAN_POINT ( 'NONE',  ( -113.2380736150634419, -292.2653605256031710, -274.0644277253857126 ) ) ;
#80066=CARTESIAN_POINT ( 'NONE',  ( 34.05115000947299109, -292.6929597509662244, -254.5884493212009545 ) ) ;
#80067=CARTESIAN_POINT ( 'NONE',  ( -6.950009051545092298, -288.1715633920741197, -341.0568289601474135 ) ) ;
#80069=CARTESIAN_POINT ( 'NONE',  ( -25.02084843196000463, -293.4728433967881642, -345.8256618156088393 ) ) ;
#80070=CARTESIAN_POINT ( 'NONE',  ( -70.59343025827944018, -281.8979763391243409, -336.2597173623353797 ) ) ;
#80071=CARTESIAN_POINT ( 'NONE',  ( -42.73031733141778687, -290.9811381663828342, -344.4519477512171761 ) ) ;
#80072=CARTESIAN_POINT ( 'NONE',  ( -102.8459195714102350, -283.4866994054297038, -236.5986390201078109 ) ) ;
#80073=CARTESIAN_POINT ( 'NONE',  ( -53.78381593217402923, -284.5826540444174384, -342.0438541648820774 ) ) ;
#80074=CARTESIAN_POINT ( 'NONE',  ( -17.77270809076263447, -289.7469904409516062, -344.5896486358663537 ) ) ;
#80075=CARTESIAN_POINT ( 'NONE',  ( 2.732503666583546931, -281.0977861864713532, -209.2099361521545973 ) ) ;
#80076=CARTESIAN_POINT ( 'NONE',  ( 31.86467039748347574, -292.7715252659738780, -303.3250442930788040 ) ) ;
#80077=CARTESIAN_POINT ( 'NONE',  ( -9.612048096015215037, -289.5017284635072770, -342.0216037376170561 ) ) ;
#80078=CARTESIAN_POINT ( 'NONE',  ( -6.938468718123411705, -289.1560986677880010, -341.0518669442762416 ) ) ;
#80079=CARTESIAN_POINT ( 'NONE',  ( -91.52264768132900485, -285.4201652888505691, -221.3641974463189683 ) ) ;
#80082=CARTESIAN_POINT ( 'NONE',  ( 34.32587455301877810, -295.7292037493839985, -295.0997561477851150 ) ) ;
#80083=CARTESIAN_POINT ( 'NONE',  ( -79.22110686710806249, -294.2894965469516819, -334.3877808903540085 ) ) ;
#80084=CARTESIAN_POINT ( 'NONE',  ( -106.6635742540715057, -277.9256354349794833, -246.5858482512796570 ) ) ;
#80085=CARTESIAN_POINT ( 'NONE',  ( -38.35031144247660251, -273.5474816154490441, -193.4292675775446355 ) ) ;
#80087=CARTESIAN_POINT ( 'NONE',  ( 32.18782895935710542, -292.3556860749015982, -294.9341212905779344 ) ) ;
#80088=CARTESIAN_POINT ( 'NONE',  ( -1.247778617471408724, -276.2980201543601879, -205.7307983549780204 ) ) ;
#80089=CARTESIAN_POINT ( 'NONE',  ( -109.2892990270986502, -294.5653881061557513, -287.7788745015828340 ) ) ;
#80090=CARTESIAN_POINT ( 'NONE',  ( 35.29853326424126436, -294.6192967123104722, -259.8479358909592065 ) ) ;
#80091=CARTESIAN_POINT ( 'NONE',  ( 32.92140940047527664, -294.3541533903462550, -249.2740717177885870 ) ) ;
#80093=CARTESIAN_POINT ( 'NONE',  ( -108.6156135490662251, -294.2440151454694615, -294.2369989424300343 ) ) ;
#80095=CARTESIAN_POINT ( 'NONE',  ( -75.30720031495870614, -275.5466224910248343, -205.6200262841623498 ) ) ;
#80096=CARTESIAN_POINT ( 'NONE',  ( -107.9820024032772068, -291.7478721366301784, -251.0386920719878106 ) ) ;
#80097=EDGE_CURVE ( 'NONE', #55253, #38497, #86590, .T. ) ;
#80098=CARTESIAN_POINT ( 'NONE',  ( -66.05754485226840700, -295.7719048644179907, -337.4989444934502671 ) ) ;
#80100=CARTESIAN_POINT ( 'NONE',  ( -111.6724978246811872, -280.3737956413369261, -282.7441433713780725 ) ) ;
#80101=CARTESIAN_POINT ( 'NONE',  ( -113.7404504103645593, -277.1858059388442257, -274.4267331729777197 ) ) ;
#80102=CARTESIAN_POINT ( 'NONE',  ( 11.72703642815687353, -274.0611899324190972, -211.0840483693015415 ) ) ;
#80103=CARTESIAN_POINT ( 'NONE',  ( -37.56899974487552640, -281.1349018589069146, -344.8134499908030648 ) ) ;
#80104=CARTESIAN_POINT ( 'NONE',  ( -68.32835065984754408, -278.0517704925619000, -200.7317423997556887 ) ) ;
#80105=CARTESIAN_POINT ( 'NONE',  ( -74.08888430577559348, -277.5648361328918554, -204.7892270330569033 ) ) ;
#80106=CARTESIAN_POINT ( 'NONE',  ( -58.02765650272269227, -296.4640526458672980, -199.8392441719955457 ) ) ;
#80107=CARTESIAN_POINT ( 'NONE',  ( 20.48984560591109272, -276.8932556611515565, -222.5865882084174530 ) ) ;
#80109=CARTESIAN_POINT ( 'NONE',  ( -92.40845807965781944, -287.8548443730286408, -321.8762068854688891 ) ) ;
#80110=CARTESIAN_POINT ( 'NONE',  ( -38.92017453879579847, -289.0714432507294305, -347.3449371820171905 ) ) ;
#80111=CARTESIAN_POINT ( 'NONE',  ( -32.81898540040753431, -276.1091532378074476, -195.3177966745486742 ) ) ;
#80112=CARTESIAN_POINT ( 'NONE',  ( -58.39681337701149033, -295.7791764750614334, -198.5508775564273378 ) ) ;
#80113=CARTESIAN_POINT ( 'NONE',  ( -111.3387315033606342, -283.4893621971894504, -291.0637305812189766 ) ) ;
#80115=CARTESIAN_POINT ( 'NONE',  ( -109.5929642193935081, -282.2926494110877798, -290.5268970055794853 ) ) ;
#80117=CARTESIAN_POINT ( 'NONE',  ( 36.03827137829312477, -292.3885319432327492, -273.5212894810681519 ) ) ;
#80118=CARTESIAN_POINT ( 'NONE',  ( -111.5432735277459670, -282.7207125640397294, -268.1268434742939917 ) ) ;
#80121=CARTESIAN_POINT ( 'NONE',  ( 14.29817831523303973, -290.7778141399049332, -215.9706445410839990 ) ) ;
#80122=CARTESIAN_POINT ( 'NONE',  ( 38.94829797198683252, -279.9909570234822809, -267.1064333782526319 ) ) ;
#80123=CARTESIAN_POINT ( 'NONE',  ( -18.79644827916364136, -278.4094885963600632, -341.7930019487720301 ) ) ;
#80124=CARTESIAN_POINT ( 'NONE',  ( -99.03363885297461877, -286.3646196544299301, -224.8633195040349904 ) ) ;
#80125=CARTESIAN_POINT ( 'NONE',  ( -27.83655209068037450, -286.1762213677894238, -197.9825841428427964 ) ) ;
#80126=CARTESIAN_POINT ( 'NONE',  ( -106.8145108695952814, -279.6553779793200647, -294.7828827014006947 ) ) ;
#80127=CARTESIAN_POINT ( 'NONE',  ( -108.7666267651937062, -279.5642426102505738, -254.4581768557627868 ) ) ;
#80128=CARTESIAN_POINT ( 'NONE',  ( -108.7727410404889241, -286.2567375100544496, -293.2640244154836751 ) ) ;
#80131=CARTESIAN_POINT ( 'NONE',  ( -110.9738579476551195, -271.0862022382013947, -270.3424529284315554 ) ) ;
#80132=CARTESIAN_POINT ( 'NONE',  ( -110.3463837949087747, -296.0771999330336257, -294.8420527524519912 ) ) ;
#80133=CARTESIAN_POINT ( 'NONE',  ( 11.20367353736895843, -290.3561906234255616, -327.1321578213385237 ) ) ;
#80135=CARTESIAN_POINT ( 'NONE',  ( -37.37352853689063181, -282.5519495502701375, -190.3611179825600175 ) ) ;
#80136=CARTESIAN_POINT ( 'NONE',  ( -53.68115742273778324, -278.7676869999617111, -195.3767049647952092 ) ) ;
#80137=CARTESIAN_POINT ( 'NONE',  ( 23.35053209991907863, -291.3313906738401329, -224.2647721550184201 ) ) ;
#80139=CARTESIAN_POINT ( 'NONE',  ( 35.64977178790378076, -289.2060730198949727, -280.5997311065902409 ) ) ;
#80140=CARTESIAN_POINT ( 'NONE',  ( -101.7039054191189393, -280.8059205225195001, -233.8168907828803924 ) ) ;
#80141=CARTESIAN_POINT ( 'NONE',  ( 38.98795499193628444, -288.9203820230122233, -265.8350665710804037 ) ) ;
#80142=CARTESIAN_POINT ( 'NONE',  ( -111.8568656840711384, -286.4372592247268017, -279.3219226463848486 ) ) ;
#80143=CARTESIAN_POINT ( 'NONE',  ( -74.09498055748265699, -277.6933367224073095, -338.0384902650253593 ) ) ;
#80145=CARTESIAN_POINT ( 'NONE',  ( -55.67375228488625538, -295.8352728631091395, -197.9489255922306370 ) ) ;
#80146=CARTESIAN_POINT ( 'NONE',  ( 38.06326802820722577, -291.7033188634103453, -275.9573157861938171 ) ) ;
#80147=CARTESIAN_POINT ( 'NONE',  ( -59.30011135599711025, -279.6088395333754306, -196.5584880779663877 ) ) ;
#80148=CARTESIAN_POINT ( 'NONE',  ( -46.35179952655523294, -275.7970394122343123, -196.6747312622376853 ) ) ;
#80150=CARTESIAN_POINT ( 'NONE',  ( 35.77081079830085031, -295.8376638359844719, -253.6410175316879361 ) ) ;
#80152=CARTESIAN_POINT ( 'NONE',  ( -96.13753662277146361, -271.4471393242510544, -222.2053487180667446 ) ) ;
#80154=CARTESIAN_POINT ( 'NONE',  ( -67.32581511905647176, -279.1556679286080680, -203.7221206800453501 ) ) ;
#80155=CARTESIAN_POINT ( 'NONE',  ( 34.34473886076967375, -276.4138413316737797, -243.3599479537965919 ) ) ;
#80156=AXIS2_PLACEMENT_3D ( 'NONE', #70701, #84872, #6772 ) ;
#80157=CARTESIAN_POINT ( 'NONE',  ( -37.84461360083788151, -299.4710052982822504, -196.7736054746696368 ) ) ;
#80158=CARTESIAN_POINT ( 'NONE',  ( -114.1199427897994241, -283.5799343416538250, -272.8296707813632338 ) ) ;
#80159=CARTESIAN_POINT ( 'NONE',  ( 31.43502135199491931, -289.6747800674957602, -297.8442249922160272 ) ) ;
#80160=CARTESIAN_POINT ( 'NONE',  ( -107.1466815574292042, -298.4705546874687911, -239.4087817870976664 ) ) ;
#80161=CARTESIAN_POINT ( 'NONE',  ( -26.29642376908139312, -299.3926162173195848, -193.7559832543641676 ) ) ;
#80162=CARTESIAN_POINT ( 'NONE',  ( 35.86628479080598453, -295.7527175164066762, -285.9345904869593937 ) ) ;
#80163=CARTESIAN_POINT ( 'NONE',  ( -10.33738327588876160, -280.6989166955122528, -340.2071184104029271 ) ) ;
#80164=CARTESIAN_POINT ( 'NONE',  ( -57.27717137448740203, -271.8138865034761693, -198.3737510935451098 ) ) ;
#80165=CARTESIAN_POINT ( 'NONE',  ( -75.72159048767646539, -287.1493804845475211, -204.4715962858715557 ) ) ;
#80166=CARTESIAN_POINT ( 'NONE',  ( -76.04354887463524904, -288.5028806387017539, -332.6218036277110741 ) ) ;
#80167=CARTESIAN_POINT ( 'NONE',  ( 7.008222688674750955, -59.14221034369032992, -354.5349928849817047 ) ) ;
#80169=CARTESIAN_POINT ( 'NONE',  ( -99.54077770306204798, -289.7193030951328865, -225.9777760355230782 ) ) ;
#80170=CARTESIAN_POINT ( 'NONE',  ( 27.04710791906520839, -287.6895065801194846, -304.9095252768789237 ) ) ;
#80171=ORIENTED_EDGE ( 'NONE', *, *, #79023, .T. ) ;
#80172=CARTESIAN_POINT ( 'NONE',  ( -109.6902236168863567, -285.9540316929830510, -244.9213133778100087 ) ) ;
#80173=CARTESIAN_POINT ( 'NONE',  ( -85.11587065588825851, -278.0662452395932860, -325.6523288780661574 ) ) ;
#80174=CARTESIAN_POINT ( 'NONE',  ( 26.24434694608633478, -291.9042219353692644, -227.3921933452214432 ) ) ;
#80175=CARTESIAN_POINT ( 'NONE',  ( -8.069993360068568933, -283.3302103268970882, -341.5265158149848617 ) ) ;
#80176=CARTESIAN_POINT ( 'NONE',  ( 36.65413941805682185, -282.8369669917644273, -251.7245012111826270 ) ) ;
#80177=CARTESIAN_POINT ( 'NONE',  ( -41.56373212361046399, -283.4371014809008216, -347.2764170675583841 ) ) ;
#80178=CARTESIAN_POINT ( 'NONE',  ( 17.07573733919547365, -281.1890097332741902, -221.6699484925040906 ) ) ;
#80179=CARTESIAN_POINT ( 'NONE',  ( -107.6853268924600258, -262.6636886874907191, -317.6917322938085704 ) ) ;
#80180=CARTESIAN_POINT ( 'NONE',  ( -72.49338645575330986, -279.5186622439703683, -336.4390797906424950 ) ) ;
#80181=CARTESIAN_POINT ( 'NONE',  ( 137.8887718377702924, 180.7638570233321502, -240.9316500215461474 ) ) ;
#80182=CARTESIAN_POINT ( 'NONE',  ( -103.4369591716781400, -253.6469098985514847, -324.2723498539693878 ) ) ;
#80183=CARTESIAN_POINT ( 'NONE',  ( -96.40569239111900401, -272.3535803324389803, -227.1023580666451380 ) ) ;
#80184=CARTESIAN_POINT ( 'NONE',  ( 30.84729256903519712, -292.5984107922258772, -234.6123205805411374 ) ) ;
#80185=CARTESIAN_POINT ( 'NONE',  ( -61.98066181902706973, -183.2303757086580163, -358.9352458450196082 ) ) ;
#80186=CARTESIAN_POINT ( 'NONE',  ( -49.62345859354491040, -272.5836358764456122, -194.7930461374557467 ) ) ;
#80187=CARTESIAN_POINT ( 'NONE',  ( -110.2122471344940635, -288.7986271683684549, -282.1165168015188556 ) ) ;
#80188=CARTESIAN_POINT ( 'NONE',  ( -91.28884199037489111, -297.6895109085813260, -321.4309179702657389 ) ) ;
#80189=CARTESIAN_POINT ( 'NONE',  ( 16.38283578654633033, -289.5844050553387206, -320.5845556226929034 ) ) ;
#80191=ORIENTED_EDGE ( 'NONE', *, *, #22848, .T. ) ;
#80192=CARTESIAN_POINT ( 'NONE',  ( 0.4351883256169691294, -295.5028322673572347, -337.2023468688740877 ) ) ;
#80193=CARTESIAN_POINT ( 'NONE',  ( -65.12242340855516431, -286.1715795532335278, -202.7334520378003049 ) ) ;
#80194=CARTESIAN_POINT ( 'NONE',  ( -107.7880932781080645, -271.8616918610850917, -239.9151886549811650 ) ) ;
#80195=CARTESIAN_POINT ( 'NONE',  ( 39.55002562315474535, -294.3542157417048770, -270.2998611162381621 ) ) ;
#80196=CARTESIAN_POINT ( 'NONE',  ( 38.00036713489024010, -293.8485377182907996, -254.7049132343567237 ) ) ;
#80197=CARTESIAN_POINT ( 'NONE',  ( -44.30231890668056849, -292.1284859796155615, -197.6429084690335003 ) ) ;
#80199=CARTESIAN_POINT ( 'NONE',  ( -107.8322266577674640, -274.8251853420545103, -243.0066827198599242 ) ) ;
#80200=CARTESIAN_POINT ( 'NONE',  ( 37.51436423037964829, -274.5523336267168020, -286.6882126927003469 ) ) ;
#80202=CARTESIAN_POINT ( 'NONE',  ( -98.52360622794620326, -278.6824386950880807, -223.6888146327250411 ) ) ;
#80203=CARTESIAN_POINT ( 'NONE',  ( 35.63577074479621842, -273.8075329434725518, -259.2882534756913628 ) ) ;
#80204=CARTESIAN_POINT ( 'NONE',  ( -67.19592490814873997, -274.7309592246189709, -203.3925201564745180 ) ) ;
#80205=CARTESIAN_POINT ( 'NONE',  ( -59.55839499149977456, -274.6986576994674465, -200.5238773939100554 ) ) ;
#80206=CARTESIAN_POINT ( 'NONE',  ( -30.59351236175934829, -299.7354243006657839, -194.1593107214988549 ) ) ;
#80207=CARTESIAN_POINT ( 'NONE',  ( 37.50083769667960354, -273.6899737794864222, -279.5724096451319838 ) ) ;
#80208=CARTESIAN_POINT ( 'NONE',  ( -61.03837610465626540, -296.0193187307580729, -339.5693759385610520 ) ) ;
#80209=CARTESIAN_POINT ( 'NONE',  ( -20.73269188929812046, -293.4095991504188987, -342.1040560909966644 ) ) ;
#80211=CARTESIAN_POINT ( 'NONE',  ( -62.38003365465612404, -277.8615380069998082, -343.1676974463954366 ) ) ;
#80213=CARTESIAN_POINT ( 'NONE',  ( -36.73820218885698097, -274.2266232278939242, -197.3511976062692383 ) ) ;
#80214=CARTESIAN_POINT ( 'NONE',  ( -113.4152973157573285, -283.1346413437733531, -278.4916827234015955 ) ) ;
#80215=CARTESIAN_POINT ( 'NONE',  ( -99.25539156025034515, -299.1289719503383253, -227.7154516038609700 ) ) ;
#80217=CARTESIAN_POINT ( 'NONE',  ( -95.88903143520013828, -284.3638118189613806, -226.4884416997613528 ) ) ;
#80218=CARTESIAN_POINT ( 'NONE',  ( -106.4525652776491285, -277.1426240698747279, -243.7287745173469489 ) ) ;
#80219=CARTESIAN_POINT ( 'NONE',  ( -68.30170890889883140, -276.0417101773569470, -337.1346427323746298 ) ) ;
#80220=AXIS2_PLACEMENT_3D ( 'NONE', #53237, #68391, #66998 ) ;
#80221=CARTESIAN_POINT ( 'NONE',  ( -63.64575781744154170, -285.3950444189775340, -340.6511832451976147 ) ) ;
#80222=CARTESIAN_POINT ( 'NONE',  ( -13.95336164956255054, -275.5675725956606357, -200.7901748558544170 ) ) ;
#80224=CARTESIAN_POINT ( 'NONE',  ( 36.10898713535917182, -274.2093581135291060, -290.6936308663386512 ) ) ;
#80226=CARTESIAN_POINT ( 'NONE',  ( 0.4301328398136732845, -282.5539307350748572, -205.3148149127621593 ) ) ;
#80228=CARTESIAN_POINT ( 'NONE',  ( -67.94045614871654948, -287.5737903070487391, -201.2598868122478279 ) ) ;
#80230=CARTESIAN_POINT ( 'NONE',  ( 36.66769178160954112, -291.7089882812107362, -282.5883829289818436 ) ) ;
#80232=CARTESIAN_POINT ( 'NONE',  ( -110.6796442498127959, -271.3090536678539593, -264.8599703506379228 ) ) ;
#80233=CARTESIAN_POINT ( 'NONE',  ( -104.6667555136829151, -289.1069088302418209, -239.0848906720252387 ) ) ;
#80234=CARTESIAN_POINT ( 'NONE',  ( -111.6667267435858832, -264.5695759149226092, -294.5014218916285245 ) ) ;
#80236=CARTESIAN_POINT ( 'NONE',  ( -71.61258491579592089, -287.9765811947996212, -338.5389311694946173 ) ) ;
#80237=CARTESIAN_POINT ( 'NONE',  ( -91.16915077849236582, -283.5396100526684222, -216.7273639724238876 ) ) ;
#80238=CARTESIAN_POINT ( 'NONE',  ( 14.35140715528836708, -283.7336158201786702, -322.8084264783296362 ) ) ;
#80239=CARTESIAN_POINT ( 'NONE',  ( -64.10494413017759996, -284.2132807828363070, -338.4517230435340593 ) ) ;
#80240=CARTESIAN_POINT ( 'NONE',  ( -108.3078535115005820, -292.2034030775747055, -295.8575675835909919 ) ) ;
#80241=CARTESIAN_POINT ( 'NONE',  ( 9.494115164424695053, -275.0098740238670985, -209.2697871955946596 ) ) ;
#80242=CARTESIAN_POINT ( 'NONE',  ( -20.83524963685109199, -286.9218768133200115, -344.1497659931614521 ) ) ;
#80243=CARTESIAN_POINT ( 'NONE',  ( 36.58585895124687681, -275.2799926308721297, -248.6407251089134434 ) ) ;
#80244=CARTESIAN_POINT ( 'NONE',  ( 18.32361299801210563, -296.2279029757397097, -320.1118729048590126 ) ) ;
#80246=CARTESIAN_POINT ( 'NONE',  ( 39.58706461736021254, -296.0519495502702512, -270.3284710469133074 ) ) ;
#80247=CARTESIAN_POINT ( 'NONE',  ( -37.55868560374530318, -281.7397839320220214, -343.8664639022123310 ) ) ;
#80249=CARTESIAN_POINT ( 'NONE',  ( -67.00903156837358665, -275.4399410922380298, -339.4254204402751611 ) ) ;
#80250=CARTESIAN_POINT ( 'NONE',  ( -33.36573434224945345, -296.5010222906605009, -194.1621739645735829 ) ) ;
#80251=CARTESIAN_POINT ( 'NONE',  ( 25.45890628494019126, -275.4144418074108671, -307.7773778457732305 ) ) ;
#80252=CARTESIAN_POINT ( 'NONE',  ( -49.82504212435136282, -293.4102987234782063, -197.6809758967185928 ) ) ;
#80253=CARTESIAN_POINT ( 'NONE',  ( 34.44475985742116819, -294.3028045848624288, -255.8658562906545058 ) ) ;
#80254=CARTESIAN_POINT ( 'NONE',  ( -97.41018203397366904, -286.9089084554425426, -227.0988654818618784 ) ) ;
#80255=CARTESIAN_POINT ( 'NONE',  ( 38.91544896830002642, -295.0482065447483251, -275.9776170493406084 ) ) ;
#80256=CARTESIAN_POINT ( 'NONE',  ( 23.64606455416303632, -295.4866709973297247, -316.5540918351017012 ) ) ;
#80257=CARTESIAN_POINT ( 'NONE',  ( -101.2135388009997996, -296.8685677401465455, -235.0144317301369199 ) ) ;
#80258=CARTESIAN_POINT ( 'NONE',  ( -69.59562228236789849, -291.4768901239034449, -338.0714211808935943 ) ) ;
#80259=CARTESIAN_POINT ( 'NONE',  ( -76.75607058193615728, -283.7308030991761143, -336.5705545799483502 ) ) ;
#80260=CARTESIAN_POINT ( 'NONE',  ( -64.99184638603904318, -295.7737370410942503, -199.9860472655927310 ) ) ;
#80261=CARTESIAN_POINT ( 'NONE',  ( -4.772018107890872329, -286.3027026627996179, -200.5885172166640587 ) ) ;
#80262=CARTESIAN_POINT ( 'NONE',  ( -59.66336925509197187, -279.3226060761432450, -341.5902544928593443 ) ) ;
#80263=CARTESIAN_POINT ( 'NONE',  ( -96.07450831871780395, -283.9616337113311602, -226.3430790909038137 ) ) ;
#80264=CARTESIAN_POINT ( 'NONE',  ( 36.14345053613208592, -285.7445636061790424, -285.3588939529307140 ) ) ;
#80265=CARTESIAN_POINT ( 'NONE',  ( -35.34445786816251456, -278.2165280338551838, -194.6097177489625096 ) ) ;
#80266=CARTESIAN_POINT ( 'NONE',  ( -104.1716275211822733, -250.7505522545870349, -322.2422935457555582 ) ) ;
#80267=CARTESIAN_POINT ( 'NONE',  ( -74.74623378463078893, -285.0472553362163808, -207.6005467327343581 ) ) ;
#80268=CARTESIAN_POINT ( 'NONE',  ( 30.36364230890859872, -282.2908167408970712, -234.4151928515386203 ) ) ;
#80269=CARTESIAN_POINT ( 'NONE',  ( -40.34160123200027925, -288.1477208693448802, -347.0802271950327622 ) ) ;
#80270=CARTESIAN_POINT ( 'NONE',  ( 7.783877076245437010, -278.0478822781354893, -331.8277832818928346 ) ) ;
#80271=CARTESIAN_POINT ( 'NONE',  ( -70.07472619770953770, -278.7894997382234692, -339.5263640227139490 ) ) ;
#80272=CARTESIAN_POINT ( 'NONE',  ( -94.78954032507844829, -279.0207439628527482, -225.2994000223949342 ) ) ;
#80273=CARTESIAN_POINT ( 'NONE',  ( -67.75013453554379339, -275.6310344586611336, -202.1769304475502054 ) ) ;
#80274=CARTESIAN_POINT ( 'NONE',  ( 13.27847622797138705, -292.7375319914993952, -212.3387279449019900 ) ) ;
#80275=CARTESIAN_POINT ( 'NONE',  ( 28.46896854776603902, -286.0431605781566304, -305.6960873448949201 ) ) ;
#80276=CARTESIAN_POINT ( 'NONE',  ( -35.00556872179647883, -293.6811223464127352, -194.1839204647555448 ) ) ;
#80277=CARTESIAN_POINT ( 'NONE',  ( 34.07343665507487174, -292.6906166228977781, -286.9724706225809427 ) ) ;
#80278=CARTESIAN_POINT ( 'NONE',  ( 3.824808897341764435, -294.1474630673001229, -330.6720292786783375 ) ) ;
#80279=CARTESIAN_POINT ( 'NONE',  ( -113.8031090717472438, -291.5492016854806820, -276.9408130151417708 ) ) ;
#80280=CARTESIAN_POINT ( 'NONE',  ( 15.32707242521286872, -281.4719112464981663, -219.5947011091182901 ) ) ;
#80281=CARTESIAN_POINT ( 'NONE',  ( -96.74633864127601157, -272.2658958494441208, -221.7205606208881363 ) ) ;
#80282=CARTESIAN_POINT ( 'NONE',  ( -1.840397811864377342, -289.2457177282461771, -338.5738024391012573 ) ) ;
#80283=CARTESIAN_POINT ( 'NONE',  ( -104.6970875109252148, -282.2360210423176454, -305.1679800931440809 ) ) ;
#80284=CARTESIAN_POINT ( 'NONE',  ( 3.172617539209466653, -288.8573406899253087, -335.8784775628997750 ) ) ;
#80285=CARTESIAN_POINT ( 'NONE',  ( -33.24171314383555398, -286.4383409313013544, -197.4053330546549887 ) ) ;
#80287=CARTESIAN_POINT ( 'NONE',  ( -64.81841035795852690, -181.8926033596262926, -360.5284399092209924 ) ) ;
#80288=CARTESIAN_POINT ( 'NONE',  ( -62.93877720064744352, -182.6451360637343271, -358.5784724557518075 ) ) ;
#80290=CARTESIAN_POINT ( 'NONE',  ( -81.37693647595384050, -278.6332960281381474, -211.8723474750057107 ) ) ;
#80291=CARTESIAN_POINT ( 'NONE',  ( -110.2721489523059972, -277.5766063470999825, -262.4339883428488065 ) ) ;
#80292=CARTESIAN_POINT ( 'NONE',  ( 39.29668692297522625, -275.1216153680238676, -262.5867002607046174 ) ) ;
#80293=CARTESIAN_POINT ( 'NONE',  ( -87.47509635287066487, -230.6792793315559607, -345.4377264683223530 ) ) ;
#80295=CARTESIAN_POINT ( 'NONE',  ( -42.37299311322092166, -278.5646001980651363, -194.1161680902108344 ) ) ;
#80296=CARTESIAN_POINT ( 'NONE',  ( -48.60111788454638315, -281.2163224418533218, -344.1518512235516027 ) ) ;
#80297=CARTESIAN_POINT ( 'NONE',  ( -11.38204671525669376, -296.4788136624466119, -341.8317268058464151 ) ) ;
#80298=CARTESIAN_POINT ( 'NONE',  ( -87.97775539916428045, -291.8132438612482815, -217.6226238143446494 ) ) ;
#80299=CARTESIAN_POINT ( 'NONE',  ( -18.36219085221994263, -287.4874003300274694, -341.4142086671831748 ) ) ;
#80300=CARTESIAN_POINT ( 'NONE',  ( -92.10230355117157330, -273.9460803960664066, -216.3741834594142688 ) ) ;
#80301=CARTESIAN_POINT ( 'NONE',  ( -103.7194740258367887, -297.1300117867306767, -239.8586718505176805 ) ) ;
#80304=CARTESIAN_POINT ( 'NONE',  ( -97.44606076710093134, -281.0945497193244478, -224.5494222949722598 ) ) ;
#80306=CARTESIAN_POINT ( 'NONE',  ( 25.39372497046981536, -282.1107776778738412, -232.3353101186652339 ) ) ;
#80307=CARTESIAN_POINT ( 'NONE',  ( -90.60256909669053016, -279.5540528342153834, -324.6312179729694094 ) ) ;
#80308=CARTESIAN_POINT ( 'NONE',  ( -8.683498064682357409, -272.9138382001413561, -202.4140126628049359 ) ) ;
#80311=CARTESIAN_POINT ( 'NONE',  ( 28.35915969007604787, -275.8326241957810794, -230.4152778563501442 ) ) ;
#80312=CARTESIAN_POINT ( 'NONE',  ( 30.06914310202902030, -277.9870224728589392, -303.3546937354441866 ) ) ;
#80315=CARTESIAN_POINT ( 'NONE',  ( 26.91591439077548387, -284.0586696708265890, -309.8220395367054039 ) ) ;
#80316=CARTESIAN_POINT ( 'NONE',  ( -65.37940793661114469, -290.8732011608630614, -202.7717755022696622 ) ) ;
#80318=CARTESIAN_POINT ( 'NONE',  ( 1.477395180076321868, -285.9052545169872701, -203.9651495795492053 ) ) ;
#80319=CARTESIAN_POINT ( 'NONE',  ( -107.9593265488379075, -282.5023039711295496, -292.5224548648868677 ) ) ;
#80320=CARTESIAN_POINT ( 'NONE',  ( -59.13984719061074458, -281.9144330792287860, -340.7013610447855285 ) ) ;
#80321=CARTESIAN_POINT ( 'NONE',  ( 35.42437760287097603, -282.6262815073617389, -260.3802753046105636 ) ) ;
#80322=CARTESIAN_POINT ( 'NONE',  ( -107.2918065740294793, -270.9055020896462338, -243.1631020823736833 ) ) ;
#80323=CARTESIAN_POINT ( 'NONE',  ( -92.86275204797011895, -282.2320775502694801, -322.5707998812669075 ) ) ;
#80324=CARTESIAN_POINT ( 'NONE',  ( -105.3420330841699695, -298.1365789501898576, -301.9989966015293703 ) ) ;
#80325=CARTESIAN_POINT ( 'NONE',  ( -69.85551414817977900, -280.5543560961490925, -204.7251239632608986 ) ) ;
#80326=CARTESIAN_POINT ( 'NONE',  ( -110.5793482524169349, -286.7690747077533047, -253.4414451513140136 ) ) ;
#80328=CARTESIAN_POINT ( 'NONE',  ( 21.96236683196131168, -294.8338512104769507, -223.5180015283165744 ) ) ;
#80329=CARTESIAN_POINT ( 'NONE',  ( -36.46774208992923860, -275.0410765128344792, -345.3688393543887969 ) ) ;
#80330=CARTESIAN_POINT ( 'NONE',  ( -3.141807029913269655, -287.8091394849486164, -339.1836080373892059 ) ) ;
#80331=CARTESIAN_POINT ( 'NONE',  ( -0.8434956176400330019, -290.9452581690881630, -206.2035051943412043 ) ) ;
#80332=CARTESIAN_POINT ( 'NONE',  ( -109.7749611134550065, -277.0730410365456464, -282.8720863332231374 ) ) ;
#80333=CARTESIAN_POINT ( 'NONE',  ( -95.75989057272919069, -294.0566091649648115, -316.1670183553590618 ) ) ;
#80335=CARTESIAN_POINT ( 'NONE',  ( -25.34497988736165652, -293.5233098302275607, -197.8018994146434579 ) ) ;
#80336=CARTESIAN_POINT ( 'NONE',  ( -20.25526795762937127, -276.7662352645559167, -195.3538533559490702 ) ) ;
#80338=CARTESIAN_POINT ( 'NONE',  ( -74.28778874486029338, -294.0136180977058871, -337.1862663831909117 ) ) ;
#80339=CARTESIAN_POINT ( 'NONE',  ( 28.95526563748203230, -289.5866738515966858, -302.7826038102975872 ) ) ;
#80340=CARTESIAN_POINT ( 'NONE',  ( -96.51527554341554094, -288.1442830426971682, -318.0519917138868777 ) ) ;
#80341=CARTESIAN_POINT ( 'NONE',  ( -13.07659988956628005, -290.1558734470841614, -339.8347088428878919 ) ) ;
#80343=CARTESIAN_POINT ( 'NONE',  ( -98.97229980445470687, -290.8108568269145735, -309.7853606563520543 ) ) ;
#80345=CARTESIAN_POINT ( 'NONE',  ( 23.83440981576210760, -289.3742880678108804, -316.4641796154584199 ) ) ;
#80346=CARTESIAN_POINT ( 'NONE',  ( -93.71421849647849456, -277.2646032648693222, -220.3556585084283199 ) ) ;
#80347=CARTESIAN_POINT ( 'NONE',  ( -42.43289429708828919, -280.3228697736262802, -193.5508059569522459 ) ) ;
#80348=VECTOR ( 'NONE', #88868, 1000.000000000000000 ) ;
#80349=CARTESIAN_POINT ( 'NONE',  ( -77.47786862572245070, -279.1962863488473658, -204.6120280759215859 ) ) ;
#80350=CARTESIAN_POINT ( 'NONE',  ( 36.54199945121559523, -285.3826938225514596, -257.1757657295149215 ) ) ;
#80352=CARTESIAN_POINT ( 'NONE',  ( -96.58339880190602855, -277.3099660019990438, -225.6042841602528028 ) ) ;
#80353=CARTESIAN_POINT ( 'NONE',  ( -101.2281313779566432, -282.0248365376669994, -309.6488329771750614 ) ) ;
#80354=CARTESIAN_POINT ( 'NONE',  ( -47.42491241558246173, -156.7151974593914190, -362.7999322911606441 ) ) ;
#80355=CARTESIAN_POINT ( 'NONE',  ( -82.15488251693280120, -276.1310803426380858, -332.1226467461781340 ) ) ;
#80356=CARTESIAN_POINT ( 'NONE',  ( -112.0554627081022403, -283.6897415074474225, -253.0594939968741528 ) ) ;
#80357=CARTESIAN_POINT ( 'NONE',  ( -108.6946458389171966, -273.5677800443384058, -254.1945207536275859 ) ) ;
#80358=CARTESIAN_POINT ( 'NONE',  ( -52.44703789090385726, -275.2877491416678026, -195.4042534402165927 ) ) ;
#80359=CARTESIAN_POINT ( 'NONE',  ( 20.85120060232780759, -275.8385673865425929, -314.4709104490390814 ) ) ;
#80360=CARTESIAN_POINT ( 'NONE',  ( -53.55764435794566936, -297.2602238324482755, -343.6405008410101232 ) ) ;
#80361=CARTESIAN_POINT ( 'NONE',  ( -57.28885219312510912, -289.4692056267678595, -344.7876629160396078 ) ) ;
#80362=CARTESIAN_POINT ( 'NONE',  ( 5.390398428577372059, -278.7054708981266913, -208.0451332852020698 ) ) ;
#80363=CARTESIAN_POINT ( 'NONE',  ( -58.93665064041741175, -291.6135693750293854, -196.4513208183290942 ) ) ;
#80364=CARTESIAN_POINT ( 'NONE',  ( -15.79382446902911497, -287.8253293910272532, -340.4076635772473196 ) ) ;
#80365=CARTESIAN_POINT ( 'NONE',  ( -5.431338903037021382, -290.4718106567270866, -202.4882257529098410 ) ) ;
#80368=CARTESIAN_POINT ( 'NONE',  ( -102.9034113917912805, -289.6232649502455843, -302.6047290959142515 ) ) ;
#80370=CARTESIAN_POINT ( 'NONE',  ( 24.50656396498728640, -287.8875341668129408, -224.8901113722191383 ) ) ;
#80371=CARTESIAN_POINT ( 'NONE',  ( -37.37352853689063181, -288.5519495502701375, -200.3611179825600459 ) ) ;
#80372=CARTESIAN_POINT ( 'NONE',  ( 0.4142989221714316606, -293.6206321889089850, -337.2141490228852376 ) ) ;
#80373=CARTESIAN_POINT ( 'NONE',  ( -33.06943442094281949, -284.3145973165848659, -346.7616416610520673 ) ) ;
#80374=CARTESIAN_POINT ( 'NONE',  ( -65.09125361108934271, -285.5126587298330492, -202.7872229992557038 ) ) ;
#80375=CARTESIAN_POINT ( 'NONE',  ( 35.59764983834237739, -276.9906568814339494, -279.7729882763896399 ) ) ;
#80376=CARTESIAN_POINT ( 'NONE',  ( 34.32238351275083943, -291.8429545140094774, -291.2901540116704950 ) ) ;
#80377=CARTESIAN_POINT ( 'NONE',  ( -46.21163202100608913, -272.7320417375804027, -197.5019743382674164 ) ) ;
#80379=CARTESIAN_POINT ( 'NONE',  ( 202.9737475146022803, 296.4636489462809550, -68.70538243550777224 ) ) ;
#80380=CARTESIAN_POINT ( 'NONE',  ( 33.39546151682874608, -293.6072486570630531, -300.8601426496741738 ) ) ;
#80381=CARTESIAN_POINT ( 'NONE',  ( -30.42129283807700801, -288.0603702630351677, -196.1916943921049494 ) ) ;
#80382=CARTESIAN_POINT ( 'NONE',  ( -95.34636527920996230, -298.3129103428891540, -220.1126156360013795 ) ) ;
#80383=CARTESIAN_POINT ( 'NONE',  ( 16.04324499545989369, -287.4859282217960867, -220.4032817418305967 ) ) ;
#80384=CARTESIAN_POINT ( 'NONE',  ( -72.74286869506777009, -276.5680991823698491, -338.4902217201118333 ) ) ;
#80385=CARTESIAN_POINT ( 'NONE',  ( -8.418668381705955994, -295.3348644015867421, -341.6689911046485690 ) ) ;
#80386=CARTESIAN_POINT ( 'NONE',  ( 15.80238528944281562, -286.4492852364213036, -324.4341564320301927 ) ) ;
#80387=CARTESIAN_POINT ( 'NONE',  ( 39.20462864995405994, -293.7773845494611464, -261.7240737623294535 ) ) ;
#80388=CARTESIAN_POINT ( 'NONE',  ( -37.55427151558518517, -292.3827367420563519, -197.3278360403185445 ) ) ;
#80391=CARTESIAN_POINT ( 'NONE',  ( 173.9547979362525894, 240.3581496378278928, -177.1551773923532380 ) ) ;
#80392=CARTESIAN_POINT ( 'NONE',  ( -23.92699244239541656, -287.7405087752162558, -195.1891291902018395 ) ) ;
#80393=CARTESIAN_POINT ( 'NONE',  ( -111.2586520408596868, -288.4809262143061801, -234.7283546768995564 ) ) ;
#80395=CARTESIAN_POINT ( 'NONE',  ( -114.1086100312523115, -277.9569603705388658, -265.8717605420122254 ) ) ;
#80396=CARTESIAN_POINT ( 'NONE',  ( 23.59186286994720660, -282.9602990343876741, -226.9200161494502765 ) ) ;
#80397=CARTESIAN_POINT ( 'NONE',  ( -75.66117004219593412, -209.4785753004333060, -356.0246882555991306 ) ) ;
#80398=CARTESIAN_POINT ( 'NONE',  ( -110.3575498293441512, -283.4139577534669456, -247.6600260010800127 ) ) ;
#80399=CARTESIAN_POINT ( 'NONE',  ( -69.39985025201343660, -287.5572103574889979, -337.5443689650706460 ) ) ;
#80400=CARTESIAN_POINT ( 'NONE',  ( -52.32491076153355181, -275.7228227631503614, -196.0390550074943690 ) ) ;
#80401=CARTESIAN_POINT ( 'NONE',  ( -63.10703266408297907, -298.1998052001035262, -201.9399374625336634 ) ) ;
#80402=CARTESIAN_POINT ( 'NONE',  ( 31.99980827499022951, -292.5606009983550848, -294.8649601378671719 ) ) ;
#80403=CARTESIAN_POINT ( 'NONE',  ( -82.47973865649710490, -278.3022659419894467, -332.6176057095522651 ) ) ;
#80404=CARTESIAN_POINT ( 'NONE',  ( -40.50576614797915909, -277.0930097537486176, -343.3049794409141100 ) ) ;
#80405=CARTESIAN_POINT ( 'NONE',  ( 32.26669578359336299, -276.2168914236885371, -238.0452073168526965 ) ) ;
#80406=CARTESIAN_POINT ( 'NONE',  ( -101.8444841358155060, -276.9249240674079147, -311.9415778431463195 ) ) ;
#80407=CARTESIAN_POINT ( 'NONE',  ( 121.2562179576807182, 149.7689830916746132, -263.4557525059072987 ) ) ;
#80408=CARTESIAN_POINT ( 'NONE',  ( 37.31200593526440201, -273.6510444178789498, -278.0757982587296624 ) ) ;
#80409=CARTESIAN_POINT ( 'NONE',  ( -111.0584898532366793, -298.2334702563796895, -250.0547052613120229 ) ) ;
#80411=CARTESIAN_POINT ( 'NONE',  ( 120.8395553409046528, -299.5541904835127980, -195.3611179825600175 ) ) ;
#80413=CARTESIAN_POINT ( 'NONE',  ( 197.2116108777964030, 281.1590520725322335, -110.1526527170710921 ) ) ;
#80415=CARTESIAN_POINT ( 'NONE',  ( -35.94129136253315693, -287.1497999163134409, -197.0653818867000666 ) ) ;
#80416=CARTESIAN_POINT ( 'NONE',  ( -95.48033407271157103, -285.6444370434724647, -319.3084668643841155 ) ) ;
#80417=CARTESIAN_POINT ( 'NONE',  ( -6.966591636280974775, -285.8101783584715463, -203.8549245842454525 ) ) ;
#80418=CARTESIAN_POINT ( 'NONE',  ( -109.6672316798495501, -277.1443828610991318, -255.6192592588039076 ) ) ;
#80419=CARTESIAN_POINT ( 'NONE',  ( -83.54530099275037003, -285.5535512368696800, -328.5312171824938332 ) ) ;
#80420=CARTESIAN_POINT ( 'NONE',  ( -36.98573078637099343, -278.5365660730943773, -196.6686418364928954 ) ) ;
#80421=CARTESIAN_POINT ( 'NONE',  ( 16.76856215522951032, -277.3384903137818469, -319.8399865519692753 ) ) ;
#80423=CARTESIAN_POINT ( 'NONE',  ( -38.08927566288137001, -274.5348830603441002, -197.3034039977275143 ) ) ;
#80425=CARTESIAN_POINT ( 'NONE',  ( 32.25049177970687708, -282.7743620575975569, -303.0608178681232516 ) ) ;
#80426=CARTESIAN_POINT ( 'NONE',  ( 38.36614193868619083, -282.2169607911520188, -284.1401498912176748 ) ) ;
#80429=CARTESIAN_POINT ( 'NONE',  ( 36.17248540290382408, -289.1795047701587009, -252.0316332790257263 ) ) ;
#80430=CARTESIAN_POINT ( 'NONE',  ( -69.16753465296453385, -288.1469122262101337, -339.9485386121825741 ) ) ;
#80431=CARTESIAN_POINT ( 'NONE',  ( -105.1153225178908457, -295.3810106964807574, -297.9172032399425234 ) ) ;
#80433=CARTESIAN_POINT ( 'NONE',  ( -16.64606417490007573, -291.6613192706734026, -196.3003089214249428 ) ) ;
#80434=CARTESIAN_POINT ( 'NONE',  ( 35.68588608369223181, -285.8979943897359135, -260.1043834399056891 ) ) ;
#80435=CARTESIAN_POINT ( 'NONE',  ( -13.14256136205505321, -289.9357123768817814, -339.6542070136081293 ) ) ;
#80436=CARTESIAN_POINT ( 'NONE',  ( 35.78497577281001440, -290.2662352645559167, -287.0191576251351080 ) ) ;
#80437=CARTESIAN_POINT ( 'NONE',  ( 4.464181403716226626, -290.4882716861552012, -332.6288376780019576 ) ) ;
#80438=CARTESIAN_POINT ( 'NONE',  ( -107.1065809924027832, -288.1882506233327490, -298.3412863548136897 ) ) ;
#80439=CARTESIAN_POINT ( 'NONE',  ( -104.8190044365329783, -285.8757709481660640, -241.7663236748392137 ) ) ;
#80440=CARTESIAN_POINT ( 'NONE',  ( -94.28903256405652655, -293.2310981013047808, -221.2799465756962149 ) ) ;
#80441=CARTESIAN_POINT ( 'NONE',  ( 82.14777765880957361, -299.6392946510901538, -193.3583333091573024 ) ) ;
#80443=CARTESIAN_POINT ( 'NONE',  ( -4.223111377502405617, -300.3838190910971093, -194.7903730022934212 ) ) ;
#80444=CARTESIAN_POINT ( 'NONE',  ( 26.99219641010665072, -281.2236307810478593, -305.2000542853050433 ) ) ;
#80445=CARTESIAN_POINT ( 'NONE',  ( -97.54190663980156728, -281.9413254717118775, -315.0929387312118024 ) ) ;
#80446=CARTESIAN_POINT ( 'NONE',  ( 4.131521613627292311, -293.7060280716325451, -335.1086144417380979 ) ) ;
#80447=CARTESIAN_POINT ( 'NONE',  ( -58.11061667493238048, -296.1791441561043143, -199.5438000516386978 ) ) ;
#80448=CARTESIAN_POINT ( 'NONE',  ( 36.04941310175368585, -273.4699264072118012, -257.8330058180659421 ) ) ;
#80449=CARTESIAN_POINT ( 'NONE',  ( -39.19745702385484520, -299.3435906741805752, -196.8789062610658789 ) ) ;
#80451=CARTESIAN_POINT ( 'NONE',  ( -58.58974257309292710, -293.5629331337668191, -343.3713931510915245 ) ) ;
#80452=CARTESIAN_POINT ( 'NONE',  ( 21.00137245474618908, -295.6037587686863048, -315.2310679839309273 ) ) ;
#80454=CARTESIAN_POINT ( 'NONE',  ( -45.09771127264434654, -295.9555775853328328, -343.1609055890218656 ) ) ;
#80456=CARTESIAN_POINT ( 'NONE',  ( -70.32309218439492327, -283.6397327715861820, -202.6068960799756269 ) ) ;
#80457=CARTESIAN_POINT ( 'NONE',  ( -110.2122864278408088, -296.6094678515987653, -266.0162759452346677 ) ) ;
#80458=CARTESIAN_POINT ( 'NONE',  ( -90.43813906124488256, -283.7787744412349298, -326.1995223562259412 ) ) ;
#80459=CARTESIAN_POINT ( 'NONE',  ( -33.11439856564233253, -284.9194796525828792, -345.8156675511369826 ) ) ;
#80460=CARTESIAN_POINT ( 'NONE',  ( 39.55676283843872199, -287.1621116446310680, -265.8238749039458639 ) ) ;
#80461=CARTESIAN_POINT ( 'NONE',  ( -49.97374396222253523, -289.8905829047055818, -196.5490323371649026 ) ) ;
#80462=CARTESIAN_POINT ( 'NONE',  ( -114.2830456889115283, -277.8852448426526394, -271.5984660748050601 ) ) ;
#80463=CARTESIAN_POINT ( 'NONE',  ( -20.25526795762938548, -280.3380690714490129, -345.3683826091709648 ) ) ;
#80465=CARTESIAN_POINT ( 'NONE',  ( 2.676288913461658314, -285.3971049422937085, -208.8331482667363446 ) ) ;
#80466=CARTESIAN_POINT ( 'NONE',  ( -114.0809738918028415, -289.4618034756450129, -271.2115513902590465 ) ) ;
#80468=CARTESIAN_POINT ( 'NONE',  ( -84.48844452273480954, -279.1118058660972565, -330.5597836848743327 ) ) ;
#80469=CARTESIAN_POINT ( 'NONE',  ( 10.14190292920483571, -292.4217283055657504, -328.9408569670604834 ) ) ;
#80470=CARTESIAN_POINT ( 'NONE',  ( 35.44972627992955694, -281.3032196759601220, -276.7572149369767658 ) ) ;
#80471=CARTESIAN_POINT ( 'NONE',  ( -65.60152216666924119, -295.5783124372812836, -342.0020279719682890 ) ) ;
#80472=CARTESIAN_POINT ( 'NONE',  ( -21.26604080751098280, -284.3366451853988224, -196.5309928806887854 ) ) ;
#80473=CARTESIAN_POINT ( 'NONE',  ( -97.00133783835995871, -281.1745431884944537, -224.8899053083866022 ) ) ;
#80474=CARTESIAN_POINT ( 'NONE',  ( -61.10079790909031772, -294.4269101495706877, -339.6890607983842187 ) ) ;
#80478=CARTESIAN_POINT ( 'NONE',  ( 21.80409003338201757, -282.9050155244781308, -224.8033104702516596 ) ) ;
#80479=CARTESIAN_POINT ( 'NONE',  ( -92.24105611647941316, -295.3722227420502691, -318.5695109638613758 ) ) ;
#80481=CARTESIAN_POINT ( 'NONE',  ( -37.30987171927208834, -271.5523547857346784, -195.3611179825600175 ) ) ;
#80482=CARTESIAN_POINT ( 'NONE',  ( -31.26262375507214131, -273.3242338649308749, -193.7501905062934782 ) ) ;
#80484=CARTESIAN_POINT ( 'NONE',  ( -110.2455214899932798, -290.4465169825947441, -265.7335031654978934 ) ) ;
#80486=CARTESIAN_POINT ( 'NONE',  ( -107.8964668889480265, -280.3513288828779082, -249.0836030836581187 ) ) ;
#80487=CARTESIAN_POINT ( 'NONE',  ( -63.61031775373006525, -275.3041149511859089, -201.3808152747057250 ) ) ;
#80488=CARTESIAN_POINT ( 'NONE',  ( -10.95968650386789456, -284.3141344996183193, -341.9044519121607664 ) ) ;
#80489=CARTESIAN_POINT ( 'NONE',  ( 22.90196310605353247, -280.9283076389849612, -312.2876196893815859 ) ) ;
#80490=CARTESIAN_POINT ( 'NONE',  ( -10.51552069001263767, -278.7023282810374099, -340.3993699997536737 ) ) ;
#80492=CARTESIAN_POINT ( 'NONE',  ( -83.57839670604047910, -273.2711561646557357, -208.7219258140593183 ) ) ;
#80493=CARTESIAN_POINT ( 'NONE',  ( -30.70241951479907172, -294.0568993822982407, -196.2177828088900924 ) ) ;
#80497=CARTESIAN_POINT ( 'NONE',  ( 37.13855748948093094, -291.8692051104629286, -284.3234284192116661 ) ) ;
#80498=CARTESIAN_POINT ( 'NONE',  ( 0.6498149643088227956, -274.0813040891083006, -207.9541213986141202 ) ) ;
#80500=CARTESIAN_POINT ( 'NONE',  ( 21.66073268931555873, -294.4165452876623590, -221.9728892809098397 ) ) ;
#80501=CARTESIAN_POINT ( 'NONE',  ( 35.78497577281001440, -284.2662352645559167, -287.0191576251351080 ) ) ;
#80502=CARTESIAN_POINT ( 'NONE',  ( 20.07086434238075512, -294.0667192088826596, -219.6283270696731620 ) ) ;
#80503=CARTESIAN_POINT ( 'NONE',  ( 25.04882278313685617, -288.9919255906511353, -228.9460324083932221 ) ) ;
#80504=CARTESIAN_POINT ( 'NONE',  ( 35.36177123535527045, -273.7807801538256740, -288.1416578014884635 ) ) ;
#80505=CARTESIAN_POINT ( 'NONE',  ( -95.56432010041648084, -279.8296776350105119, -316.7650966909973249 ) ) ;
#80506=CARTESIAN_POINT ( 'NONE',  ( 29.68062272051770023, -292.0633109964564937, -302.8731578813580541 ) ) ;
#80507=CARTESIAN_POINT ( 'NONE',  ( -64.32493405691835164, -281.5643069343833531, -199.5088151790409086 ) ) ;
#80509=CARTESIAN_POINT ( 'NONE',  ( -7.248640754685577114, -282.3129547156637500, -336.9067467155135773 ) ) ;
#80510=CARTESIAN_POINT ( 'NONE',  ( -2.542737627392792632, -281.5811468724717770, -202.0052132104664224 ) ) ;
#80511=CARTESIAN_POINT ( 'NONE',  ( 19.47861533819587265, -281.0490526915993428, -321.8143843649933160 ) ) ;
#80512=CARTESIAN_POINT ( 'NONE',  ( 16.79780885321362405, -277.2457933745729406, -324.8571691315373187 ) ) ;
#80513=CARTESIAN_POINT ( 'NONE',  ( 16.48004871398853410, -277.8245700654148322, -324.5267599171917254 ) ) ;
#80514=CARTESIAN_POINT ( 'NONE',  ( 17.40634833298267736, -290.6948066931273047, -313.9805196606274080 ) ) ;
#80516=CARTESIAN_POINT ( 'NONE',  ( -100.8494858809941945, -275.0852220125138956, -230.7784251220282954 ) ) ;
#80517=CARTESIAN_POINT ( 'NONE',  ( -92.79931105088246568, -292.3120855462549343, -222.4165722550149553 ) ) ;
#80518=CARTESIAN_POINT ( 'NONE',  ( -57.05837417821064150, -275.3276975731592415, -342.4085511733431417 ) ) ;
#80519=CARTESIAN_POINT ( 'NONE',  ( -83.66655920297384341, -293.1868952341234262, -210.0620601716347551 ) ) ;
#80520=CARTESIAN_POINT ( 'NONE',  ( -44.30166299510289463, -291.3105246390647380, -197.5403758345906908 ) ) ;
#80521=CARTESIAN_POINT ( 'NONE',  ( 32.80619832535118974, -287.4638201614991431, -301.9649032878892854 ) ) ;
#80523=CARTESIAN_POINT ( 'NONE',  ( 37.19062703920061352, -291.9140051033854775, -253.4637887561008824 ) ) ;
#80524=CARTESIAN_POINT ( 'NONE',  ( -74.21397431897129593, -281.9504627172444202, -334.3480382853597916 ) ) ;
#80525=CARTESIAN_POINT ( 'NONE',  ( -89.51258808471089878, -291.6574094978146832, -323.1727069473811866 ) ) ;
#80526=CARTESIAN_POINT ( 'NONE',  ( -108.7699837978218227, -282.7949836016989593, -288.4914253758695963 ) ) ;
#80527=CARTESIAN_POINT ( 'NONE',  ( 5.195047542884161373, -281.9563291684947330, -210.4289181696981075 ) ) ;
#80528=CARTESIAN_POINT ( 'NONE',  ( -82.70392661974192094, -290.5967950665985313, -332.2892103158422401 ) ) ;
#80529=CARTESIAN_POINT ( 'NONE',  ( -37.01433908642785298, -280.5487093557175626, -197.3003126446141380 ) ) ;
#80530=CARTESIAN_POINT ( 'NONE',  ( -53.29158176090530219, -290.6470509080520515, -195.3828751425093913 ) ) ;
#80531=CARTESIAN_POINT ( 'NONE',  ( 39.19284466788963073, -288.2622599756758177, -262.9626194424529331 ) ) ;
#80532=CARTESIAN_POINT ( 'NONE',  ( -9.579682989452575015, -289.1912931772486672, -342.1162384104836178 ) ) ;
#80533=CARTESIAN_POINT ( 'NONE',  ( -98.10824280512076712, -285.2803906610940885, -229.9083393933848072 ) ) ;
#80536=CARTESIAN_POINT ( 'NONE',  ( 29.81855179686944268, -295.8723563734035338, -305.4297084771415598 ) ) ;
#80537=CARTESIAN_POINT ( 'NONE',  ( -112.1266786164127041, -295.0338279995000335, -286.5012935480532974 ) ) ;
#80538=CARTESIAN_POINT ( 'NONE',  ( -59.27685380260552961, -276.4019323726130324, -340.2342707734032956 ) ) ;
#80539=CARTESIAN_POINT ( 'NONE',  ( -97.26169597338578399, -296.5475338491443722, -222.1645736553807069 ) ) ;
#80540=CARTESIAN_POINT ( 'NONE',  ( 35.89370717058314852, -292.1450562789697187, -279.0109597219382636 ) ) ;
#80541=CARTESIAN_POINT ( 'NONE',  ( -110.0367799803427573, -294.9738275315411897, -256.3869132325944520 ) ) ;
#80543=CARTESIAN_POINT ( 'NONE',  ( 11.18187833525152719, -293.9468005860555309, -215.2243293110636841 ) ) ;
#80544=CARTESIAN_POINT ( 'NONE',  ( 35.51573438171101316, -294.7444306034954593, -278.9330883976203381 ) ) ;
#80546=CARTESIAN_POINT ( 'NONE',  ( -52.93441530482945012, -293.2512535407890368, -343.9459628040423809 ) ) ;
#80547=CARTESIAN_POINT ( 'NONE',  ( -98.39224404850024541, -297.9596389803091938, -313.9469477613181425 ) ) ;
#80548=CARTESIAN_POINT ( 'NONE',  ( -100.5008205084786255, -290.9847986763157905, -307.5329838529258382 ) ) ;
#80550=CARTESIAN_POINT ( 'NONE',  ( -47.79186814010511597, -295.5218504549019940, -342.6819182620483843 ) ) ;
#80552=CARTESIAN_POINT ( 'NONE',  ( -111.1126357630462991, -280.7292592624842200, -254.9281716746444317 ) ) ;
#80553=CARTESIAN_POINT ( 'NONE',  ( -39.55609598073227318, -278.7097562860465132, -193.8733526945460142 ) ) ;
#80556=CARTESIAN_POINT ( 'NONE',  ( -105.5147294886371014, -272.3616035552637413, -234.6686622686278270 ) ) ;
#80557=CARTESIAN_POINT ( 'NONE',  ( 29.43217052193039862, -280.0706172615243190, -303.3803670117515026 ) ) ;
#80558=CARTESIAN_POINT ( 'NONE',  ( -50.77833853402099606, -278.2831164257214027, -195.3551371415321682 ) ) ;
#80559=CARTESIAN_POINT ( 'NONE',  ( -97.93452628516635627, -277.1574277938487967, -225.8586463041476122 ) ) ;
#80561=CARTESIAN_POINT ( 'NONE',  ( -69.45802370942078596, -296.3051561188211735, -204.2567668449932512 ) ) ;
#80562=CARTESIAN_POINT ( 'NONE',  ( -107.3696834841678367, -274.9030493279105940, -243.3659817668374217 ) ) ;
#80564=CARTESIAN_POINT ( 'NONE',  ( -93.46899604827929409, -289.2692449370394456, -220.0805704832913534 ) ) ;
#80565=CARTESIAN_POINT ( 'NONE',  ( -99.87026735700776214, -289.9563016343895470, -315.3189756387700982 ) ) ;
#80566=CARTESIAN_POINT ( 'NONE',  ( 28.33301635610003544, -277.0655372037653024, -233.6910553124743899 ) ) ;
#80567=CARTESIAN_POINT ( 'NONE',  ( 98.59996038885898884, -297.7573711738884299, -195.5742745502984405 ) ) ;
#80568=CARTESIAN_POINT ( 'NONE',  ( -93.79414022174815102, -284.4612531227237469, -218.1556073756473779 ) ) ;
#80570=CARTESIAN_POINT ( 'NONE',  ( 37.61795415412644417, -279.5995653411679882, -274.0665912484985824 ) ) ;
#80573=CARTESIAN_POINT ( 'NONE',  ( -25.32906956490525374, -291.0034657668256273, -197.9019878005229600 ) ) ;
#80574=CARTESIAN_POINT ( 'NONE',  ( -95.06784649677790355, -283.3410888418707714, -223.6659595435774577 ) ) ;
#80577=CARTESIAN_POINT ( 'NONE',  ( -2.690176148231683939, -290.5102143201916078, -203.8459126714049319 ) ) ;
#80578=CARTESIAN_POINT ( 'NONE',  ( -104.9967143010387360, -279.7586346608056260, -299.9719555851846167 ) ) ;
#80579=CARTESIAN_POINT ( 'NONE',  ( -63.76060060907820315, -284.5941626205424768, -342.2641806131185263 ) ) ;
#80580=CARTESIAN_POINT ( 'NONE',  ( -38.31388983956673400, -272.1199058179613530, -194.8073685777292781 ) ) ;
#80581=CARTESIAN_POINT ( 'NONE',  ( -46.72486963953097217, -285.9298474866923812, -197.9158943556960537 ) ) ;
#80582=CARTESIAN_POINT ( 'NONE',  ( 25.77191610591306059, -276.4598782102235646, -232.4200678694771511 ) ) ;
#80583=CARTESIAN_POINT ( 'NONE',  ( 20.15570014322869241, -276.9919311133270412, -315.6212204323905439 ) ) ;
#80584=CARTESIAN_POINT ( 'NONE',  ( -112.3537271438698042, -286.5208734590051449, -272.8100192037657621 ) ) ;
#80585=ORIENTED_EDGE ( 'NONE', *, *, #73503, .F. ) ;
#80587=CARTESIAN_POINT ( 'NONE',  ( -107.1672644957429270, -295.9700871516866982, -302.8170968650683221 ) ) ;
#80588=CARTESIAN_POINT ( 'NONE',  ( 21.62482275452285307, -288.9015482929277141, -224.5921767046817763 ) ) ;
#80590=CARTESIAN_POINT ( 'NONE',  ( 108.6256185021308909, -297.2649936051623740, -190.4191791630918544 ) ) ;
#80591=CARTESIAN_POINT ( 'NONE',  ( -86.59563202631936463, -278.3068472571135317, -211.5080469909619296 ) ) ;
#80592=CARTESIAN_POINT ( 'NONE',  ( -36.36790730807192773, -290.4640483067564105, -194.1544403441316433 ) ) ;
#80593=CARTESIAN_POINT ( 'NONE',  ( -104.1218797046931996, -286.4905413017955880, -239.0773581735443543 ) ) ;
#80594=CARTESIAN_POINT ( 'NONE',  ( -57.40919467121199915, -281.5497210430205541, -199.1201910233922092 ) ) ;
#80595=CARTESIAN_POINT ( 'NONE',  ( 36.80065962568925642, -288.7444315330823770, -251.8809452291229718 ) ) ;
#80596=CARTESIAN_POINT ( 'NONE',  ( 37.70437488935201031, -283.5645577177655241, -271.3144373270855567 ) ) ;
#80597=CARTESIAN_POINT ( 'NONE',  ( -99.64851363520514838, -278.1183205137967889, -315.6257852840058149 ) ) ;
#80598=CARTESIAN_POINT ( 'NONE',  ( -41.94514764665698436, -296.0139505274502767, -195.8583994094566378 ) ) ;
#80599=CARTESIAN_POINT ( 'NONE',  ( -38.16777731414562425, -279.8753885375685400, -193.3655492722977840 ) ) ;
#80601=CARTESIAN_POINT ( 'NONE',  ( -94.74842352585828564, -275.0683620204079034, -223.2739041625046070 ) ) ;
#80603=CARTESIAN_POINT ( 'NONE',  ( -95.99890600148557951, -287.6948066931273615, -223.6242672951989618 ) ) ;
#80604=CARTESIAN_POINT ( 'NONE',  ( -43.93223171177390896, -272.2099253949742774, -194.6081887851420618 ) ) ;
#80606=CARTESIAN_POINT ( 'NONE',  ( -76.84986633076367468, -279.0153687307999917, -208.8427506613836044 ) ) ;
#80608=CARTESIAN_POINT ( 'NONE',  ( 21.43587133717164050, -277.4217040808248953, -319.4855092007605890 ) ) ;
#80609=CARTESIAN_POINT ( 'NONE',  ( -61.17005598676182387, -282.4127575109083068, -343.3894364868161801 ) ) ;
#80610=CARTESIAN_POINT ( 'NONE',  ( -15.53194433218923898, -290.5262876513946821, -341.1416826281522390 ) ) ;
#80611=CARTESIAN_POINT ( 'NONE',  ( -57.22785902341170328, -299.3203508725534903, -196.6364723243882509 ) ) ;
#80613=CARTESIAN_POINT ( 'NONE',  ( -112.5020922378360240, -297.9440762879806357, -255.4975068239502889 ) ) ;
#80614=EDGE_CURVE ( 'NONE', #75524, #16725, #64933, .T. ) ;
#80615=CARTESIAN_POINT ( 'NONE',  ( 24.46114235158401584, -296.1260809147493092, -312.6470023915463230 ) ) ;
#80616=CARTESIAN_POINT ( 'NONE',  ( 19.37016060382411098, -278.8735348475181013, -221.5173336865785529 ) ) ;
#80618=CARTESIAN_POINT ( 'NONE',  ( -31.17934293839923754, -272.1504588927260215, -195.9581829050052022 ) ) ;
#80619=CARTESIAN_POINT ( 'NONE',  ( -89.35521443607908054, -286.9348496448824335, -214.6023984822353157 ) ) ;
#80620=CARTESIAN_POINT ( 'NONE',  ( -68.90346522408979979, -288.3975569416243729, -336.5281872749503123 ) ) ;
#80621=CARTESIAN_POINT ( 'NONE',  ( 169.5516713374554456, 231.4314716580894071, -192.4310804009363665 ) ) ;
#80623=CARTESIAN_POINT ( 'NONE',  ( -3.339366624424855434, -287.1868004975563622, -338.8040455191342062 ) ) ;
#80624=CARTESIAN_POINT ( 'NONE',  ( 34.30407757348636011, -287.4057453997950233, -284.5314100344209010 ) ) ;
#80626=CARTESIAN_POINT ( 'NONE',  ( -4.917186391078216978, -287.5488524038057108, -200.8618847489759105 ) ) ;
#80627=CARTESIAN_POINT ( 'NONE',  ( -40.50243445195970082, -277.4262370723741356, -343.3262915105309503 ) ) ;
#80628=CARTESIAN_POINT ( 'NONE',  ( 39.19265033448239421, -292.5436661972052548, -276.0300475646976111 ) ) ;
#80629=CARTESIAN_POINT ( 'NONE',  ( 25.85130039774165311, -282.7834178363546584, -314.2015992173868995 ) ) ;
#80630=CARTESIAN_POINT ( 'NONE',  ( 32.93501657957552453, -283.4556118962891560, -300.2264410652383617 ) ) ;
#80631=CARTESIAN_POINT ( 'NONE',  ( -96.25139210699917669, -284.2178077463306636, -319.9334288332771621 ) ) ;
#80632=CARTESIAN_POINT ( 'NONE',  ( 33.13287274737167110, -281.6324163675899399, -251.1972740236468837 ) ) ;
#80633=CARTESIAN_POINT ( 'NONE',  ( -54.49178911615187104, -274.7666405000204577, -345.3538533559490702 ) ) ;
#80634=CARTESIAN_POINT ( 'NONE',  ( -21.92796979628985099, -108.3679673722940890, -362.8334583402871658 ) ) ;
#80636=CARTESIAN_POINT ( 'NONE',  ( -112.1856056875244008, -280.5843480040693407, -267.8720730314923344 ) ) ;
#80637=CARTESIAN_POINT ( 'NONE',  ( 202.2089753311514926, 295.8238823582390182, -68.59691984642449825 ) ) ;
#80638=CARTESIAN_POINT ( 'NONE',  ( -40.16685237741654646, -139.4501677287193502, -361.1782757304578126 ) ) ;
#80640=CARTESIAN_POINT ( 'NONE',  ( -93.68683404902384382, -296.5602610471650564, -223.7678503208838379 ) ) ;
#80641=CARTESIAN_POINT ( 'NONE',  ( 23.97613257082112881, -293.6794421192739719, -316.8331557748318801 ) ) ;
#80642=CARTESIAN_POINT ( 'NONE',  ( 46.05136225311299114, 10.74623296475258627, -328.6500756323578685 ) ) ;
#80643=CARTESIAN_POINT ( 'NONE',  ( -48.86308555104901075, -296.4830194937312058, -194.7706940381690970 ) ) ;
#80644=CARTESIAN_POINT ( 'NONE',  ( -94.73920026989721066, -288.3030305993506204, -316.7504205760400851 ) ) ;
#80645=CARTESIAN_POINT ( 'NONE',  ( -45.19829872390753422, -297.0129904678551611, -344.2307342631454503 ) ) ;
#80646=CARTESIAN_POINT ( 'NONE',  ( -18.32988954735931841, -290.1173250778139163, -341.4055725574542066 ) ) ;
#80648=CARTESIAN_POINT ( 'NONE',  ( -11.12626039145826340, -295.6600564492915737, -342.5671606866590650 ) ) ;
#80649=CARTESIAN_POINT ( 'NONE',  ( -73.59160737361305848, -286.0495101476194577, -206.9121336901716859 ) ) ;
#80650=CARTESIAN_POINT ( 'NONE',  ( -33.34474327913569169, -296.8960777995857256, -193.7589848913696358 ) ) ;
#80652=CARTESIAN_POINT ( 'NONE',  ( 32.03576029928489532, -293.9293210171288138, -237.2083198445805010 ) ) ;
#80653=CARTESIAN_POINT ( 'NONE',  ( 38.29790953048718904, -294.2215879961315750, -284.5098473702107071 ) ) ;
#80654=CARTESIAN_POINT ( 'NONE',  ( -66.56602437012034557, -291.8250603831472745, -203.4661340366758395 ) ) ;
#80657=CARTESIAN_POINT ( 'NONE',  ( -8.267702724943189807, -276.3498943526248581, -200.5630844522248708 ) ) ;
#80658=CARTESIAN_POINT ( 'NONE',  ( 33.35305942019162728, -273.9684279267765987, -240.7238860052175085 ) ) ;
#80660=CARTESIAN_POINT ( 'NONE',  ( -17.37991209284142968, -276.3088828790554317, -344.6649127813457198 ) ) ;
#80661=CARTESIAN_POINT ( 'NONE',  ( -72.26854459626602534, -271.9822259945433416, -205.2922156131260181 ) ) ;
#80662=CARTESIAN_POINT ( 'NONE',  ( 18.34639594754544945, -274.3812704080507388, -319.4689974431610153 ) ) ;
#80663=CARTESIAN_POINT ( 'NONE',  ( 52.26321846338277766, -300.4034925610951063, -196.9452196686116849 ) ) ;
#80664=CARTESIAN_POINT ( 'NONE',  ( -32.68801561960830782, -275.0534625816939638, -197.2612632450224623 ) ) ;
#80665=CARTESIAN_POINT ( 'NONE',  ( -36.92305596632481013, -299.6574319610531916, -194.1610007473992425 ) ) ;
#80666=CARTESIAN_POINT ( 'NONE',  ( 3.982697788410620277, -272.6254278401342503, -207.2856974345233425 ) ) ;
#80667=CARTESIAN_POINT ( 'NONE',  ( -38.33536874342558320, -295.7163486224669668, -343.4562976541824924 ) ) ;
#80668=CARTESIAN_POINT ( 'NONE',  ( -42.44858803093227806, -293.6925451356875101, -343.7729332000806153 ) ) ;
#80669=DIRECTION ( 'NONE',  ( 0.000000000000000000, 0.000000000000000000, 1.000000000000000000 ) ) ;
#80670=CARTESIAN_POINT ( 'NONE',  ( 21.68744721306714851, -276.7090908225387125, -319.7077153084395036 ) ) ;
#80671=CARTESIAN_POINT ( 'NONE',  ( -34.04280338166187647, -274.2614786291991891, -197.4356952222026678 ) ) ;
#80672=CARTESIAN_POINT ( 'NONE',  ( -66.98244148497897754, -284.3565134170310102, -199.8293894821586605 ) ) ;
#80673=CARTESIAN_POINT ( 'NONE',  ( -91.36132212530594643, -297.8187481375859988, -322.6287835645019300 ) ) ;
#80675=AXIS2_PLACEMENT_3D ( 'NONE', #8363, #61827, #32935 ) ;
#80676=CARTESIAN_POINT ( 'NONE',  ( -71.24398842751128313, -284.7896357092502058, -205.5287450856548048 ) ) ;
#80677=CARTESIAN_POINT ( 'NONE',  ( -100.3183350266978948, -277.3220132211541227, -231.3800096711332799 ) ) ;
#80678=CARTESIAN_POINT ( 'NONE',  ( -93.18553236381445970, -276.4500524535504269, -318.2864903817628033 ) ) ;
#80679=CARTESIAN_POINT ( 'NONE',  ( -28.26766519831462077, -284.9373004810215662, -344.8618117954649733 ) ) ;
#80680=CARTESIAN_POINT ( 'NONE',  ( 20.15703958886026470, -276.1165621682254141, -224.7227557075171092 ) ) ;
#80682=CARTESIAN_POINT ( 'NONE',  ( 10.01279240863232367, -274.8122076995315979, -330.1276643319100117 ) ) ;
#80684=CARTESIAN_POINT ( 'NONE',  ( -6.994466967600344809, -282.4495544418196573, -201.5789260721935818 ) ) ;
#80686=CARTESIAN_POINT ( 'NONE',  ( -46.35837608101083873, -287.8587413280799296, -195.3410289967331437 ) ) ;
#80689=CARTESIAN_POINT ( 'NONE',  ( -105.5727227803703414, -288.9620752939506474, -239.1005386117919898 ) ) ;
#80691=CARTESIAN_POINT ( 'NONE',  ( -109.0121239484455060, -271.4501164827466368, -254.0947776090119419 ) ) ;
#80692=CARTESIAN_POINT ( 'NONE',  ( -103.4998016162079892, -289.1428355648584443, -236.5729113685504785 ) ) ;
#80693=CARTESIAN_POINT ( 'NONE',  ( 117.8046289747227320, 148.0164379187816053, -257.9426961570557069 ) ) ;
#80695=CARTESIAN_POINT ( 'NONE',  ( 7.511191807944600285, -286.9328762090681835, -332.1589624366116595 ) ) ;
#80696=CARTESIAN_POINT ( 'NONE',  ( 6.079041424221729883, -284.0519553649695013, -330.0359000625119847 ) ) ;
#80697=CARTESIAN_POINT ( 'NONE',  ( -113.3125630315945216, -282.8328988306882934, -267.1347769798854870 ) ) ;
#80698=CARTESIAN_POINT ( 'NONE',  ( -108.3504172742902369, -290.3287437157649720, -287.2951691591007943 ) ) ;
#80701=CARTESIAN_POINT ( 'NONE',  ( 34.90931797535003511, -282.7937461364803653, -256.3246587310170526 ) ) ;
#80702=CARTESIAN_POINT ( 'NONE',  ( -2.342442496387988626, -283.3793297680984438, -334.6222583516037048 ) ) ;
#80703=CARTESIAN_POINT ( 'NONE',  ( -69.90497682248880551, -291.4586717020156357, -338.3314535750560026 ) ) ;
#80704=CARTESIAN_POINT ( 'NONE',  ( 30.78618628518020373, -299.0497418230892208, -193.3592212852306318 ) ) ;
#80706=CARTESIAN_POINT ( 'NONE',  ( 11.46667891486397473, -286.4611437164322183, -328.0417588463044467 ) ) ;
#80707=CARTESIAN_POINT ( 'NONE',  ( -0.04544512761132132872, -274.5342885334318908, -202.9815245707586087 ) ) ;
#80708=CARTESIAN_POINT ( 'NONE',  ( -28.68065138822588978, -296.9218163533998336, -344.5539126099598093 ) ) ;
#80710=CARTESIAN_POINT ( 'NONE',  ( 35.78497577281001440, -290.2662352645559167, -287.0191576251351080 ) ) ;
#80711=CARTESIAN_POINT ( 'NONE',  ( -5.836634923200410441, -281.3139294116411975, -336.7728089953354242 ) ) ;
#80712=CARTESIAN_POINT ( 'NONE',  ( -98.18123366909019012, -275.9518301094695403, -314.5257324059594453 ) ) ;
#80713=CARTESIAN_POINT ( 'NONE',  ( -80.83913248881592040, -271.9538145460363694, -207.6019543870419284 ) ) ;
#80714=CARTESIAN_POINT ( 'NONE',  ( 25.36753299582257526, -274.3835271994092864, -232.6938536957339920 ) ) ;
#80715=CARTESIAN_POINT ( 'NONE',  ( -32.12736780972890926, -293.6392091423817874, -196.8397491205238339 ) ) ;
#80716=CIRCLE ( 'NONE', #47447, 6.338655513825452559 ) ;
#80717=CARTESIAN_POINT ( 'NONE',  ( 32.02002961880699416, -294.1802606469486250, -246.7010149481445467 ) ) ;
#80718=CARTESIAN_POINT ( 'NONE',  ( -110.4964874198071527, -286.1617758118932215, -281.9298906159953617 ) ) ;
#80719=CARTESIAN_POINT ( 'NONE',  ( 28.95532888275551997, -294.4799965604088356, -232.3701949094345309 ) ) ;
#80720=CARTESIAN_POINT ( 'NONE',  ( 19.17675958178251605, -295.5735539856111131, -322.0034272664332207 ) ) ;
#80721=CARTESIAN_POINT ( 'NONE',  ( -80.15649115309555839, -295.4836010988398698, -329.4872008391952249 ) ) ;
#80722=CARTESIAN_POINT ( 'NONE',  ( -92.03424078925327478, -291.8327591062536612, -321.7567772052939858 ) ) ;
#80723=CARTESIAN_POINT ( 'NONE',  ( -95.33333507678375440, -284.0337332961186121, -321.0165252012948258 ) ) ;
#80724=CARTESIAN_POINT ( 'NONE',  ( -112.6325156277984689, -270.7992862870522686, -261.8995235254844260 ) ) ;
#80725=CARTESIAN_POINT ( 'NONE',  ( -114.3407554914418540, -284.3902425960415030, -269.9797026784136733 ) ) ;
#80726=CARTESIAN_POINT ( 'NONE',  ( -68.70609260014886388, -279.4463236246886026, -338.1108478244917706 ) ) ;
#80727=CARTESIAN_POINT ( 'NONE',  ( -110.3880023331265789, -283.4476732166726833, -262.6933978173333344 ) ) ;
#80728=CARTESIAN_POINT ( 'NONE',  ( 18.12745533052277835, -286.2565682542181662, -320.8596755229561381 ) ) ;
#80729=CARTESIAN_POINT ( 'NONE',  ( -111.1923468024427279, -276.9068386878082038, -253.4381315162311807 ) ) ;
#80730=CARTESIAN_POINT ( 'NONE',  ( 84.09003387609358526, 83.72762891241104910, -302.5758382668069544 ) ) ;
#80731=CARTESIAN_POINT ( 'NONE',  ( -107.4121885052917946, -284.3354467313042164, -249.4947627439274243 ) ) ;
#80732=CARTESIAN_POINT ( 'NONE',  ( 27.97450754521559091, -283.2839780505913154, -310.4841881115479509 ) ) ;
#80733=CARTESIAN_POINT ( 'NONE',  ( -3.176254805997625219, -287.6707424742872945, -339.1182827741045571 ) ) ;
#80734=CARTESIAN_POINT ( 'NONE',  ( -88.65816948899072258, -279.3583210976050282, -326.6910424108231155 ) ) ;
#80735=EDGE_CURVE ( 'NONE', #47701, #72158, #79577, .T. ) ;
#80736=CARTESIAN_POINT ( 'NONE',  ( 12.39679360693573074, -277.6912109917018938, -328.4935573985345059 ) ) ;
#80737=CARTESIAN_POINT ( 'NONE',  ( -35.66067117326975477, -279.9071115699464372, -197.3680729565291756 ) ) ;
#80739=CARTESIAN_POINT ( 'NONE',  ( -3.378317565346750762, -276.4826888935253351, -203.8762101897231673 ) ) ;
#80740=CARTESIAN_POINT ( 'NONE',  ( 37.42194470148324115, -293.3216869639346669, -251.9383762810997780 ) ) ;
#80741=CARTESIAN_POINT ( 'NONE',  ( 16.36249123482662426, -284.8170321379483312, -218.2469331948977640 ) ) ;
#80742=CARTESIAN_POINT ( 'NONE',  ( -42.02536033575427155, -293.5941647697928261, -194.3051928809160245 ) ) ;
#80743=CARTESIAN_POINT ( 'NONE',  ( -69.87355327019915308, -294.4113844697831723, -336.0566627765817884 ) ) ;
#80744=CARTESIAN_POINT ( 'NONE',  ( 31.55859179288613703, -293.5423356067616396, -294.6959015195108691 ) ) ;
#80745=CARTESIAN_POINT ( 'NONE',  ( -47.71524630523616395, -293.0030092285787759, -194.3214733833709715 ) ) ;
#80746=CARTESIAN_POINT ( 'NONE',  ( 34.04174452890308089, -282.4111437847175239, -286.1185447227665009 ) ) ;
#80747=CARTESIAN_POINT ( 'NONE',  ( -9.237262086084902180, -297.3166033843284026, -193.6752382179209633 ) ) ;
#80748=CARTESIAN_POINT ( 'NONE',  ( 38.57570410709797670, -288.3609225647131780, -282.9268169659338810 ) ) ;
#80749=CARTESIAN_POINT ( 'NONE',  ( 18.85121182303647558, -280.3938182899094045, -321.2577442569548225 ) ) ;
#80750=CARTESIAN_POINT ( 'NONE',  ( 34.02432539428471614, -288.2534716252163207, -299.3585290927771894 ) ) ;
#80751=CARTESIAN_POINT ( 'NONE',  ( -59.98921508271534009, -286.0836848681150855, -200.9408215765164698 ) ) ;
#80754=CARTESIAN_POINT ( 'NONE',  ( 137.0887459190394679, 180.1851913858904766, -239.5941216051346032 ) ) ;
#80755=CARTESIAN_POINT ( 'NONE',  ( 201.7738562182570661, 292.3636489450776708, -53.99999999998410516 ) ) ;
#80756=CARTESIAN_POINT ( 'NONE',  ( -109.2890452841104292, -277.9240275538465994, -257.0877893752386854 ) ) ;
#80757=CARTESIAN_POINT ( 'NONE',  ( -110.2128643799814256, -277.3614662463560876, -278.8118533307255689 ) ) ;
#80758=CARTESIAN_POINT ( 'NONE',  ( -9.132041924864411797, -297.9041281600072466, -193.4249352461565650 ) ) ;
#80759=CARTESIAN_POINT ( 'NONE',  ( -11.13748388457448790, -93.05548120058779205, -357.1551308049848785 ) ) ;
#80760=CARTESIAN_POINT ( 'NONE',  ( -107.9611199367248560, -277.5006323421724801, -241.1805793072681752 ) ) ;
#80762=CARTESIAN_POINT ( 'NONE',  ( 23.23489877041117069, -295.9315662353751009, -316.2353992550123394 ) ) ;
#80763=CARTESIAN_POINT ( 'NONE',  ( -22.73444753245486183, -292.7365334218281419, -198.7746904067340665 ) ) ;
#80764=CARTESIAN_POINT ( 'NONE',  ( -101.4206850775283613, -297.9141795850052290, -227.9338231061404088 ) ) ;
#80765=CARTESIAN_POINT ( 'NONE',  ( -3.151777270829502431, -287.2757789271626052, -335.4735453984766309 ) ) ;
#80766=CARTESIAN_POINT ( 'NONE',  ( -111.7218282884229126, -273.4505231540948671, -250.6403448215230867 ) ) ;
#80767=CARTESIAN_POINT ( 'NONE',  ( -109.1417444117289790, -296.5440327891541870, -283.6119185539668024 ) ) ;
#80772=CARTESIAN_POINT ( 'NONE',  ( -112.6117965512912633, -280.5638836903187325, -263.1756497733751985 ) ) ;
#80774=CARTESIAN_POINT ( 'NONE',  ( -110.4679533834542724, -279.6998041295244661, -265.1864529924664566 ) ) ;
#80775=CARTESIAN_POINT ( 'NONE',  ( -86.42334322707458227, -279.4825635086385773, -328.4382755050291962 ) ) ;
#80776=CARTESIAN_POINT ( 'NONE',  ( -79.23344749411340615, -271.9556465748632945, -209.6708550135730036 ) ) ;
#80777=LINE ( 'NONE', #64298, #413 ) ;
#80778=CARTESIAN_POINT ( 'NONE',  ( 129.4467878515196162, -299.5541904835127980, -200.7046326357662167 ) ) ;
#80779=CARTESIAN_POINT ( 'NONE',  ( -62.31094260811752150, -279.8849374510551229, -201.7108436353591969 ) ) ;
#80780=CARTESIAN_POINT ( 'NONE',  ( 0.9754012281359498715, -277.3575839374287284, -337.0244654815010676 ) ) ;
#80782=CARTESIAN_POINT ( 'NONE',  ( 2.462230916218959287, -278.5192513584873382, -333.9883533326937481 ) ) ;
#80783=CARTESIAN_POINT ( 'NONE',  ( -109.1889831946827627, -276.7940754479504335, -296.5270434734528635 ) ) ;
#80784=EDGE_LOOP ( 'NONE', ( #87391, #44079, #52084, #59946, #39161 ) ) ;
#80786=CARTESIAN_POINT ( 'NONE',  ( 34.90903669404877263, -283.8085414261822734, -291.9473257305984930 ) ) ;
#80787=CARTESIAN_POINT ( 'NONE',  ( -107.5473703500983333, -290.0215945511944824, -249.7310884712448456 ) ) ;
#80788=CARTESIAN_POINT ( 'NONE',  ( -49.32065485834987584, -285.2520230882961982, -194.3481395924868025 ) ) ;
#80789=CARTESIAN_POINT ( 'NONE',  ( -107.1367117731449810, -282.4669304159499461, -295.1437363591193161 ) ) ;
#80790=CARTESIAN_POINT ( 'NONE',  ( -76.45556027577532632, -282.1608352030651190, -332.7550164340187848 ) ) ;
#80791=CARTESIAN_POINT ( 'NONE',  ( 9.964069392794204560, -284.7897193035814212, -212.8852242100739716 ) ) ;
#80792=CARTESIAN_POINT ( 'NONE',  ( -34.31221878957652649, -281.2961284327006410, -197.0139798273647784 ) ) ;
#80794=CARTESIAN_POINT ( 'NONE',  ( 17.23887642618106852, -280.6894548620743421, -323.6098032450410074 ) ) ;
#80795=CARTESIAN_POINT ( 'NONE',  ( 30.36909351505336829, -295.1264562740456086, -237.9876190257857900 ) ) ;
#80796=CARTESIAN_POINT ( 'NONE',  ( -107.2115936112030283, -278.9172058406896895, -292.0268518571219261 ) ) ;
#80797=CARTESIAN_POINT ( 'NONE',  ( -69.04340306327220844, -287.6364293456096561, -202.1926326118442887 ) ) ;
#80799=CARTESIAN_POINT ( 'NONE',  ( -98.87289171003052957, -293.0641890920890660, -226.5065097648617041 ) ) ;
#80800=CARTESIAN_POINT ( 'NONE',  ( -23.99812914350882309, -274.8816854556443445, -344.2174294559167151 ) ) ;
#80801=CARTESIAN_POINT ( 'NONE',  ( -38.92711335558434627, -288.2687405391064885, -347.1832846144802147 ) ) ;
#80802=CARTESIAN_POINT ( 'NONE',  ( -25.25825090711430221, -290.6084767101443731, -197.5050163048832133 ) ) ;
#80803=CARTESIAN_POINT ( 'NONE',  ( -104.7302311409926290, -276.8438014001201282, -299.8149630055418697 ) ) ;
#80804=CARTESIAN_POINT ( 'NONE',  ( -108.7981029369255452, -294.4301856929252494, -290.4819524438684084 ) ) ;
#80805=CARTESIAN_POINT ( 'NONE',  ( -110.4652262588898992, -291.9637926657075013, -262.9995010671385671 ) ) ;
#80806=DIRECTION ( 'NONE',  ( 0.000000000000000000, 0.000000000000000000, -1.000000000000000000 ) ) ;
#80807=CARTESIAN_POINT ( 'NONE',  ( 27.50640061612403997, -292.5639290026003891, -310.6776540298927785 ) ) ;
#80808=CARTESIAN_POINT ( 'NONE',  ( 7.395881705345527024, -288.2735091921749699, -211.6025337545028719 ) ) ;
#80809=CARTESIAN_POINT ( 'NONE',  ( -99.85980111615754140, -288.2140498186846003, -313.5521015672636054 ) ) ;
#80810=CARTESIAN_POINT ( 'NONE',  ( 22.45096607517663756, -289.5722765538042154, -313.2588100689136468 ) ) ;
#80812=CARTESIAN_POINT ( 'NONE',  ( -105.2591433654582289, -290.9901215845535489, -297.6967179592811021 ) ) ;
#80813=CARTESIAN_POINT ( 'NONE',  ( -37.65625321811246096, -297.0359238922718532, -345.7284651688788131 ) ) ;
#80815=CARTESIAN_POINT ( 'NONE',  ( -43.13687005376367978, -290.3288640853958782, -346.7445240610447854 ) ) ;
#80816=CARTESIAN_POINT ( 'NONE',  ( -110.7927256074832059, -276.7873817904935549, -253.5280058539548520 ) ) ;
#80817=CARTESIAN_POINT ( 'NONE',  ( -50.94006445514779102, -280.2162147420324914, -194.5928609149019906 ) ) ;
#80818=CARTESIAN_POINT ( 'NONE',  ( 17.21112458519271016, -280.4710883573537217, -215.9749191443662824 ) ) ;
#80819=CARTESIAN_POINT ( 'NONE',  ( -92.98848233180861200, -283.2536745904423015, -220.0012799249687134 ) ) ;
#80821=CARTESIAN_POINT ( 'NONE',  ( 7.913775325800443738, -278.8170988821121341, -211.4504393562112625 ) ) ;
#80822=CARTESIAN_POINT ( 'NONE',  ( -5.048672459209301522, -280.6269117234355122, -338.0668893420386780 ) ) ;
#80824=CARTESIAN_POINT ( 'NONE',  ( -111.7215318996356359, -277.2470775444506330, -253.3215058508797597 ) ) ;
#80825=CARTESIAN_POINT ( 'NONE',  ( -37.16722594807185232, -299.5745066800461132, -196.6648578062816455 ) ) ;
#80826=CARTESIAN_POINT ( 'NONE',  ( -88.12717539434204639, -282.6634580603832774, -327.8979222978668986 ) ) ;
#80827=CARTESIAN_POINT ( 'NONE',  ( -71.99321534080206675, -274.3847987021081281, -205.8696271848382366 ) ) ;
#80828=CARTESIAN_POINT ( 'NONE',  ( 18.92067436663976565, -300.0578547439411636, -193.8419764170976407 ) ) ;
#80829=CARTESIAN_POINT ( 'NONE',  ( 34.86320200767453059, -275.0741756914497387, -259.3893663229188178 ) ) ;
#80830=CARTESIAN_POINT ( 'NONE',  ( -73.05510320491455900, -297.5255909549920830, -336.3269203277943689 ) ) ;
#80831=CARTESIAN_POINT ( 'NONE',  ( -96.38968977502322844, -290.0535359697130389, -319.8015534905158574 ) ) ;
#80832=CARTESIAN_POINT ( 'NONE',  ( -40.91535955006486347, -278.0873946025727719, -194.8727217248486738 ) ) ;
#80834=CARTESIAN_POINT ( 'NONE',  ( -101.6827927269252996, -290.9426087811735329, -227.9662236921970759 ) ) ;
#80836=CARTESIAN_POINT ( 'NONE',  ( -53.47197783344539346, -288.3229403575269885, -341.7979613374839118 ) ) ;
#80837=CARTESIAN_POINT ( 'NONE',  ( 35.48614395923007692, -291.3218501149586359, -252.4416933766567865 ) ) ;
#80840=CARTESIAN_POINT ( 'NONE',  ( -109.3363081884106265, -290.2275803959498717, -257.6319502625115092 ) ) ;
#80842=CARTESIAN_POINT ( 'NONE',  ( 0.1583475295494594925, -287.4800369293899962, -203.3642793163164129 ) ) ;
#80843=CARTESIAN_POINT ( 'NONE',  ( 7.399455738971494334, -295.1948066931273615, -214.2051214447836571 ) ) ;
#80844=CARTESIAN_POINT ( 'NONE',  ( 6.469851476471298213, -293.5318797081282582, -333.4605390768797406 ) ) ;
#80846=CARTESIAN_POINT ( 'NONE',  ( -63.72613161114504265, -284.7042431466907715, -342.1744875436768325 ) ) ;
#80847=CARTESIAN_POINT ( 'NONE',  ( -74.71828596398320599, -285.3728699584102060, -207.6555294297379817 ) ) ;
#80848=CARTESIAN_POINT ( 'NONE',  ( 18.69521969451735899, -277.5388818947328105, -317.9122178225212565 ) ) ;
#80849=CARTESIAN_POINT ( 'NONE',  ( 34.69761165295190608, -291.8253849117466530, -289.9591906224781042 ) ) ;
#80850=AXIS2_PLACEMENT_3D ( 'NONE', #84599, #41978, #57614 ) ;
#80851=CARTESIAN_POINT ( 'NONE',  ( -2.712835635230579800, -273.3157590727560091, -205.6465736392402732 ) ) ;
#80854=CARTESIAN_POINT ( 'NONE',  ( 0.5264022157440970684, -294.2285048531094276, -337.3968205271914940 ) ) ;
#80855=CARTESIAN_POINT ( 'NONE',  ( 14.11768923642479479, -288.7012147585972457, -216.5011291933842870 ) ) ;
#80856=CARTESIAN_POINT ( 'NONE',  ( -97.15766721518704685, -296.9859163018715549, -318.3771321035365531 ) ) ;
#80857=CARTESIAN_POINT ( 'NONE',  ( -5.762117462996388717, -287.1300569388433246, -204.4183943034166475 ) ) ;
#80858=CARTESIAN_POINT ( 'NONE',  ( -110.3222376340370658, -277.9132005616436345, -246.3878397897619834 ) ) ;
#80859=CARTESIAN_POINT ( 'NONE',  ( -30.71433344388374920, -292.7851271298282541, -193.6964800947524736 ) ) ;
#80860=CARTESIAN_POINT ( 'NONE',  ( 38.34512336514053743, -285.6352227209219450, -265.9148848488836165 ) ) ;
#80861=CARTESIAN_POINT ( 'NONE',  ( 38.05074099482647654, -294.0799276647240390, -285.9085973009398458 ) ) ;
#80862=CARTESIAN_POINT ( 'NONE',  ( -7.265413793488712635, -292.7911519563569982, -203.8216222888351297 ) ) ;
#80863=CARTESIAN_POINT ( 'NONE',  ( 121.3887860922853150, -299.5541904835127980, -195.3611179825600175 ) ) ;
#80866=CARTESIAN_POINT ( 'NONE',  ( 2.363572411682822061, -288.0941586262227361, -205.1982521407357751 ) ) ;
#80867=CARTESIAN_POINT ( 'NONE',  ( 40.64545035920995986, -285.2666405000203440, -288.1938231032136741 ) ) ;
#80869=CARTESIAN_POINT ( 'NONE',  ( -8.384742108316707743, -281.5842092396390512, -337.7088770877577986 ) ) ;
#80870=CARTESIAN_POINT ( 'NONE',  ( -95.19770440732621353, -277.5315372047091955, -321.1393324097162463 ) ) ;
#80871=CARTESIAN_POINT ( 'NONE',  ( -1.099953963021016445, -282.5344932052304330, -204.8892594259328916 ) ) ;
#80872=CARTESIAN_POINT ( 'NONE',  ( -68.86288425581687989, -197.2185115433246381, -359.2771530895120122 ) ) ;
#80873=CARTESIAN_POINT ( 'NONE',  ( -100.4991487550860825, -283.6995131681854900, -227.2590439676938843 ) ) ;
#80875=CARTESIAN_POINT ( 'NONE',  ( 24.91962922687913462, -285.0125148525706322, -229.0925754941216326 ) ) ;
#80876=CARTESIAN_POINT ( 'NONE',  ( 6.500614332665397122, -276.5009111174006193, -208.5055103792745683 ) ) ;
#80877=CARTESIAN_POINT ( 'NONE',  ( -52.65410000597154294, -298.3431302024771981, -198.8702710869863495 ) ) ;
#80878=CARTESIAN_POINT ( 'NONE',  ( -5.341822208537517547, -293.3068515727523504, -336.5358187631491091 ) ) ;
#80879=CARTESIAN_POINT ( 'NONE',  ( -113.9431494924813393, -279.2953472221363995, -263.0319032181764101 ) ) ;
#80880=CARTESIAN_POINT ( 'NONE',  ( -41.85658474486650960, -277.1105909851053184, -343.2339629271970125 ) ) ;
#80881=CARTESIAN_POINT ( 'NONE',  ( -113.8735839098065412, -273.7033722426746181, -264.6629600359769370 ) ) ;
#80882=CARTESIAN_POINT ( 'NONE',  ( -112.8784203360696381, -270.8800938378385581, -296.3057481714963046 ) ) ;
#80883=CARTESIAN_POINT ( 'NONE',  ( -3.189148384620934085, -274.6009566780471687, -337.1479835168137811 ) ) ;
#80884=CARTESIAN_POINT ( 'NONE',  ( -88.19961510018092099, -297.1727374243644704, -327.4590559622506589 ) ) ;
#80887=CARTESIAN_POINT ( 'NONE',  ( -71.54095004379935574, -284.5948383734786944, -335.2042932558952089 ) ) ;
#80888=CARTESIAN_POINT ( 'NONE',  ( -110.5095964938329161, -286.0519219365333470, -290.8655798501631580 ) ) ;
#80889=CARTESIAN_POINT ( 'NONE',  ( -73.59899006222124740, -284.9059343601233536, -206.8698225293622386 ) ) ;
#80890=CARTESIAN_POINT ( 'NONE',  ( -87.65566418352666744, -276.1689209581305136, -324.3513526064785992 ) ) ;
#80891=CARTESIAN_POINT ( 'NONE',  ( -87.75050315396148903, -285.6253470096708043, -324.9274606503319092 ) ) ;
#80892=CARTESIAN_POINT ( 'NONE',  ( -66.32472241315528549, -278.1455566757566089, -202.5927044084809268 ) ) ;
#80893=CARTESIAN_POINT ( 'NONE',  ( 3.316921798269993005, -277.5710095182063242, -331.3619584366844606 ) ) ;
#80895=CARTESIAN_POINT ( 'NONE',  ( -104.4387055546949625, -273.4342340904827893, -241.3195581572348942 ) ) ;
#80897=CARTESIAN_POINT ( 'NONE',  ( 30.57429261198475601, -281.8886383253222903, -234.3091980900835836 ) ) ;
#80898=CARTESIAN_POINT ( 'NONE',  ( 29.71134787749449657, -282.5356082247352560, -308.1978949779359027 ) ) ;
#80902=CARTESIAN_POINT ( 'NONE',  ( 34.77934137657171476, -289.7092353481821192, -293.5744945686486744 ) ) ;
#80904=CARTESIAN_POINT ( 'NONE',  ( -97.00852005224960806, -296.3392132321985173, -228.0235185306095218 ) ) ;
#80905=CARTESIAN_POINT ( 'NONE',  ( -30.69779667728393591, -291.4825108423753477, -193.6979123986693594 ) ) ;
#80906=CARTESIAN_POINT ( 'NONE',  ( 26.28499433688804032, -286.5387682590465488, -307.6419447866070982 ) ) ;
#80907=CARTESIAN_POINT ( 'NONE',  ( 34.85876485693646742, -286.3139308670872083, -284.6552950761611669 ) ) ;
#80908=CARTESIAN_POINT ( 'NONE',  ( -38.89670468638797018, -290.2722369875604045, -196.3641182001636309 ) ) ;
#80909=CARTESIAN_POINT ( 'NONE',  ( -72.57804954362150340, -286.7797417549978150, -205.9610309928523009 ) ) ;
#80910=CARTESIAN_POINT ( 'NONE',  ( -112.2362121774151262, -276.5009297386895355, -274.3376379402653242 ) ) ;
#80911=CARTESIAN_POINT ( 'NONE',  ( 38.80381423493700765, -286.0030799819184040, -274.4010520032072691 ) ) ;
#80912=CARTESIAN_POINT ( 'NONE',  ( -57.25021422476851995, -287.7955695978098447, -197.9977824795448953 ) ) ;
#80913=CARTESIAN_POINT ( 'NONE',  ( -103.5533819354939311, -288.0807596484780220, -305.9425965351536547 ) ) ;
#80914=CARTESIAN_POINT ( 'NONE',  ( 29.53420116598874401, -282.8955484070024227, -300.3356754801890247 ) ) ;
#80915=CARTESIAN_POINT ( 'NONE',  ( -98.55325287289387859, -293.1441825852793954, -226.7357327266190907 ) ) ;
#80916=CARTESIAN_POINT ( 'NONE',  ( 82.16069579344274132, -298.6247067295462330, -193.5820051170746297 ) ) ;
#80918=CARTESIAN_POINT ( 'NONE',  ( -103.9951007501086053, -298.9422436401694654, -234.6601946772061353 ) ) ;
#80921=CARTESIAN_POINT ( 'NONE',  ( 18.09355462092307221, -280.0706692306564491, -222.5974153240782982 ) ) ;
#80922=CARTESIAN_POINT ( 'NONE',  ( 18.57034904698929623, -278.8559449401706729, -220.3726852480296259 ) ) ;
#80923=CARTESIAN_POINT ( 'NONE',  ( -16.56039960223472463, -293.9875738063915946, -344.3912037942455413 ) ) ;
#80924=CARTESIAN_POINT ( 'NONE',  ( -37.80733690747151599, -296.4460944566480407, -196.5625841215439209 ) ) ;
#80925=CARTESIAN_POINT ( 'NONE',  ( 34.62828102998530966, -273.8782533770864802, -289.3778477870255870 ) ) ;
#80926=CARTESIAN_POINT ( 'NONE',  ( -107.3338236263226833, -297.5701405377287188, -292.9388246761129153 ) ) ;
#80928=CARTESIAN_POINT ( 'NONE',  ( -105.0648837072402557, -294.3410257966332892, -304.9378594723468154 ) ) ;
#80929=CARTESIAN_POINT ( 'NONE',  ( 4.163563080981257158, -295.9057333466056434, -331.1286096365158187 ) ) ;
#80931=CARTESIAN_POINT ( 'NONE',  ( -50.49021521649092392, -296.0272074197996517, -342.3313776559213011 ) ) ;
#80932=DIRECTION ( 'NONE',  ( 0.000000000000000000, 1.000000000000000000, 7.202301750926674102E-15 ) ) ;
#80933=CARTESIAN_POINT ( 'NONE',  ( -105.1870544760080008, -283.0022208108266568, -237.5676019597713093 ) ) ;
#80934=CARTESIAN_POINT ( 'NONE',  ( -81.94411708228696511, -297.4251187390993891, -212.5075690501982990 ) ) ;
#80935=CARTESIAN_POINT ( 'NONE',  ( -113.1369744685507897, -284.3788108970562689, -284.2213454163775168 ) ) ;
#80936=CARTESIAN_POINT ( 'NONE',  ( 37.44947268265346452, -283.6093297445146959, -281.1126140492563650 ) ) ;
#80937=CARTESIAN_POINT ( 'NONE',  ( -46.49877174559616577, -285.6056692503037198, -193.9288451466239280 ) ) ;
#80938=CARTESIAN_POINT ( 'NONE',  ( -60.81034762864257459, -289.7468991514519416, -199.2486713137323306 ) ) ;
#80939=CARTESIAN_POINT ( 'NONE',  ( 31.98288692825982693, -272.6237833571632905, -237.0123917617630980 ) ) ;
#80941=CARTESIAN_POINT ( 'NONE',  ( 31.44203322619777552, -285.8921673213552026, -244.3322107758392860 ) ) ;
#80942=CARTESIAN_POINT ( 'NONE',  ( -99.62728815232638624, -288.8768046418859399, -315.1273152812001968 ) ) ;
#80943=DIRECTION ( 'NONE',  ( 0.000000000000000000, 0.000000000000000000, 1.000000000000000000 ) ) ;
#80944=CARTESIAN_POINT ( 'NONE',  ( -108.2334561269400126, -298.4206595650496752, -249.8477236400458992 ) ) ;
#80945=CARTESIAN_POINT ( 'NONE',  ( -105.6569804930849727, -280.4224371361070780, -236.0141575381979635 ) ) ;
#80946=CARTESIAN_POINT ( 'NONE',  ( 12.29307649831085847, -292.3858026675229667, -327.1294502709004064 ) ) ;
#80947=CARTESIAN_POINT ( 'NONE',  ( 28.16816198786099434, -281.6572348123985989, -302.7333412904417855 ) ) ;
#80948=CARTESIAN_POINT ( 'NONE',  ( -19.28522074316199664, -294.9928501384467268, -345.2689501496894309 ) ) ;
#80949=CARTESIAN_POINT ( 'NONE',  ( -40.72701110398927682, -284.0898680019321887, -194.8257700697250812 ) ) ;
#80950=CARTESIAN_POINT ( 'NONE',  ( -61.43002905117817392, -281.7395822208497407, -199.2799141292963441 ) ) ;
#80952=CARTESIAN_POINT ( 'NONE',  ( -23.48602998284878041, -293.9295517078970761, -342.3255346346486476 ) ) ;
#80953=CARTESIAN_POINT ( 'NONE',  ( -43.10984599156205377, -295.9792986177575358, -195.5314249023259947 ) ) ;
#80956=CARTESIAN_POINT ( 'NONE',  ( 10.30754250284056361, -282.6928055696701563, -212.8359783770726779 ) ) ;
#80957=CARTESIAN_POINT ( 'NONE',  ( -75.69569416502747572, -295.0863798966923923, -332.6049855037002771 ) ) ;
#80959=CARTESIAN_POINT ( 'NONE',  ( -92.05005921254146983, -294.6952119285919025, -226.6919474004047572 ) ) ;
#80960=CARTESIAN_POINT ( 'NONE',  ( -70.05371433758904232, -272.8293408454781002, -200.8191658664519252 ) ) ;
#80961=CARTESIAN_POINT ( 'NONE',  ( -91.67173919388861236, -291.0834466493888044, -221.5854032711879427 ) ) ;
#80962=CARTESIAN_POINT ( 'NONE',  ( -27.48462164438750222, -281.6996346729844731, -197.2783136474464243 ) ) ;
#80963=CARTESIAN_POINT ( 'NONE',  ( -81.56652468207778384, -275.0394463142596919, -211.2156354820562001 ) ) ;
#80964=CARTESIAN_POINT ( 'NONE',  ( -44.32538618581968137, -284.7390759999619263, -346.2932228828734083 ) ) ;
#80965=CARTESIAN_POINT ( 'NONE',  ( -91.57995490408625017, -278.0523690607897151, -220.9107163250839108 ) ) ;
#80966=CARTESIAN_POINT ( 'NONE',  ( -59.76945595974496683, -279.3428711020333139, -341.9292422769228210 ) ) ;
#80968=CARTESIAN_POINT ( 'NONE',  ( -0.04358587629538659969, -274.3676354107399789, -202.9825537491880425 ) ) ;
#80969=CARTESIAN_POINT ( 'NONE',  ( -34.83276561095786406, -294.0040718146144627, -195.9634066742511322 ) ) ;
#80973=CARTESIAN_POINT ( 'NONE',  ( -0.08783136817415880537, -292.7016166352680102, -336.3491882483041309 ) ) ;
#80974=CARTESIAN_POINT ( 'NONE',  ( 94.46225245802311576, -299.4135974027564089, -197.3478171873541669 ) ) ;
#80976=EDGE_CURVE ( 'NONE', #42078, #33611, #14721, .T. ) ;
#80977=CARTESIAN_POINT ( 'NONE',  ( -68.06750732326811715, -293.1761310821050870, -200.4996701153740162 ) ) ;
#80978=CARTESIAN_POINT ( 'NONE',  ( -85.33152481854864391, -275.9090924074130839, -210.2361428286349110 ) ) ;
#80979=CARTESIAN_POINT ( 'NONE',  ( 37.38166234488451778, -289.4890081780330888, -265.4414161113364798 ) ) ;
#80980=CARTESIAN_POINT ( 'NONE',  ( 10.82511592784155141, -274.3840315779106618, -327.6322822322093202 ) ) ;
#80981=CARTESIAN_POINT ( 'NONE',  ( 37.02415473366912835, -277.4163000128716590, -266.0313103988966077 ) ) ;
#80982=CARTESIAN_POINT ( 'NONE',  ( 37.06137684319755721, -291.6016631164964679, -268.0166922013801241 ) ) ;
#80983=CARTESIAN_POINT ( 'NONE',  ( -53.52019912407880042, -281.7073012417760651, -196.2901147211961472 ) ) ;
#80986=CARTESIAN_POINT ( 'NONE',  ( -93.44103837372750831, -283.5558013726102899, -317.1045852829162186 ) ) ;
#80987=CARTESIAN_POINT ( 'NONE',  ( -82.35370408541332665, -278.7304551895524583, -332.4530821058404513 ) ) ;
#80988=CARTESIAN_POINT ( 'NONE',  ( -33.09617432451796759, -281.7947545888164314, -346.8593749361108394 ) ) ;
#80989=CARTESIAN_POINT ( 'NONE',  ( -84.71173679581764304, -278.6278634440695896, -330.8347775141432976 ) ) ;
#80990=CARTESIAN_POINT ( 'NONE',  ( 36.92162573082385535, -277.2942806637337299, -287.9578773858711429 ) ) ;
#80991=CARTESIAN_POINT ( 'NONE',  ( -6.998514795304313196, -288.9805209788416391, -207.2794874003663779 ) ) ;
#80993=CARTESIAN_POINT ( 'NONE',  ( -105.7506846275603181, -298.1477255294961992, -301.2322638647054873 ) ) ;
#80994=CARTESIAN_POINT ( 'NONE',  ( -104.9936166230227030, -292.0105962207279049, -241.9899019872270856 ) ) ;
#80995=CARTESIAN_POINT ( 'NONE',  ( -111.9245850319576192, -276.5330386405051968, -273.4008678493808020 ) ) ;
#80996=CARTESIAN_POINT ( 'NONE',  ( -107.8497421667622405, -291.9479468211941366, -298.6911377430700441 ) ) ;
#80997=CARTESIAN_POINT ( 'NONE',  ( -9.681227136689926738, -291.7717535669419817, -202.6404911404750919 ) ) ;
#80998=CARTESIAN_POINT ( 'NONE',  ( 37.08329244450528961, -287.3041584072681189, -289.8661784538941220 ) ) ;
#80999=CARTESIAN_POINT ( 'NONE',  ( -110.7884892328630571, -283.0526842193842754, -262.6463874164611525 ) ) ;
#81000=CARTESIAN_POINT ( 'NONE',  ( -87.54761236490108445, -291.6217818917674549, -325.1138439125219293 ) ) ;
#81001=CARTESIAN_POINT ( 'NONE',  ( -73.88276017995251266, -284.0373658272128523, -206.3507153379153181 ) ) ;
#81002=CARTESIAN_POINT ( 'NONE',  ( 31.52659216117618257, -282.5256495625073399, -244.5558649205003405 ) ) ;
#81003=CARTESIAN_POINT ( 'NONE',  ( -71.79010550537037716, -290.4375569107573938, -338.9623394065972093 ) ) ;
#81004=CARTESIAN_POINT ( 'NONE',  ( -109.1025422709250989, -278.8627298746004044, -284.1519865446053927 ) ) ;
#81005=CARTESIAN_POINT ( 'NONE',  ( -39.18666668507475492, -290.8244439326350061, -193.7674419063706353 ) ) ;
#81006=CARTESIAN_POINT ( 'NONE',  ( -15.46923084645170832, -287.1309415353467216, -196.6461273896154580 ) ) ;
#81007=CARTESIAN_POINT ( 'NONE',  ( 33.98763866029031533, -288.4125120336144050, -299.3414366975588905 ) ) ;
#81008=CARTESIAN_POINT ( 'NONE',  ( -104.5983809761635115, -285.1013236576974919, -241.8491640071268023 ) ) ;
#81011=CARTESIAN_POINT ( 'NONE',  ( -36.41762190707066082, -293.9240318489935362, -194.5891269432724471 ) ) ;
#81012=CARTESIAN_POINT ( 'NONE',  ( -111.8295423015167671, -295.0164994129381171, -287.8780650214542902 ) ) ;
#81013=CARTESIAN_POINT ( 'NONE',  ( -43.23794448056239048, -276.1871791569755601, -343.3586710289284269 ) ) ;
#81014=CARTESIAN_POINT ( 'NONE',  ( -48.94640524150316452, -297.2567539731875286, -194.2901330421438217 ) ) ;
#81015=CARTESIAN_POINT ( 'NONE',  ( 21.06094800268414957, -292.6588410975414263, -315.3243851279051455 ) ) ;
#81016=CARTESIAN_POINT ( 'NONE',  ( -67.20797283515103970, -295.8949788273944819, -202.6273880238698837 ) ) ;
#81017=CARTESIAN_POINT ( 'NONE',  ( -69.20378073829436971, -292.8285407349191587, -204.2266040007081074 ) ) ;
#81018=CARTESIAN_POINT ( 'NONE',  ( 17.32019187608983657, -295.3278275698817765, -319.2298553253233422 ) ) ;
#81020=CARTESIAN_POINT ( 'NONE',  ( 34.60722761199123454, -291.8337937111373890, -292.2945376055183715 ) ) ;
#81021=CARTESIAN_POINT ( 'NONE',  ( -46.76279720659812966, -299.9328330479887086, -195.9035009737389998 ) ) ;
#81022=CARTESIAN_POINT ( 'NONE',  ( -95.94943698683739797, -290.8786930168090521, -314.2972058669748776 ) ) ;
#81023=CARTESIAN_POINT ( 'NONE',  ( -34.29606572000218279, -295.3460898357508881, -343.3187193540831572 ) ) ;
#81024=CARTESIAN_POINT ( 'NONE',  ( -15.05164067315313048, -278.7449016956053924, -342.3988109580352557 ) ) ;
#81025=CARTESIAN_POINT ( 'NONE',  ( -112.7475847567949927, -277.3997644745304001, -257.4285684779155190 ) ) ;
#81026=CARTESIAN_POINT ( 'NONE',  ( -92.09066196691415485, -272.6434640186287766, -216.3623775894970152 ) ) ;
#81027=CARTESIAN_POINT ( 'NONE',  ( 24.89974019181063625, -279.0757743414590095, -229.4353190999128174 ) ) ;
#81028=CARTESIAN_POINT ( 'NONE',  ( -112.2826064898294192, -276.7767850834315482, -284.2278717966325416 ) ) ;
#81030=CARTESIAN_POINT ( 'NONE',  ( 95.54697187129778513, -298.4345910877814845, -196.8985534675756810 ) ) ;
#81032=CARTESIAN_POINT ( 'NONE',  ( 17.35631459575653324, -275.5108287996426952, -221.7884948099801647 ) ) ;
#81034=CARTESIAN_POINT ( 'NONE',  ( -108.3248792541964036, -288.2442567293040838, -295.8101322244813787 ) ) ;
#81035=CARTESIAN_POINT ( 'NONE',  ( -65.44702332552137136, -289.4094629418118529, -342.1049131632886429 ) ) ;
#81036=CARTESIAN_POINT ( 'NONE',  ( 30.87819878916672067, -277.1372324003118024, -238.6766222048762813 ) ) ;
#81037=CARTESIAN_POINT ( 'NONE',  ( -39.18867085314754917, -296.0287923967409256, -195.5378555190710586 ) ) ;
#81038=CARTESIAN_POINT ( 'NONE',  ( -30.24001523134090874, -282.1616333731604982, -346.8707571922872148 ) ) ;
#81040=CARTESIAN_POINT ( 'NONE',  ( -7.028099366246645552, -280.6542849723426798, -338.9757737723930973 ) ) ;
#81043=CARTESIAN_POINT ( 'NONE',  ( -2.236089605140999304, -291.3226378346382148, -205.8896753515070372 ) ) ;
#81044=CARTESIAN_POINT ( 'NONE',  ( -14.15813556143607244, -284.4954930384076306, -199.7849451296545737 ) ) ;
#81047=CARTESIAN_POINT ( 'NONE',  ( 37.28808806273238474, -291.4499572040390944, -262.4146482955856641 ) ) ;
#81048=CARTESIAN_POINT ( 'NONE',  ( -76.76615179585407134, -279.1892942604593486, -332.8083330218639730 ) ) ;
#81049=CARTESIAN_POINT ( 'NONE',  ( -83.63099041918093235, -284.8761227367322135, -331.4630610348853565 ) ) ;
#81050=CARTESIAN_POINT ( 'NONE',  ( 8.653505572859097938, -272.7568014588411529, -210.4131801722226669 ) ) ;
#81051=CARTESIAN_POINT ( 'NONE',  ( -109.1930275799229548, -284.7232403703180239, -257.3916972783390520 ) ) ;
#81052=CARTESIAN_POINT ( 'NONE',  ( -18.85150736666681581, -278.2346606510798210, -341.5895370801849253 ) ) ;
#81053=CARTESIAN_POINT ( 'NONE',  ( -9.918369515986093177, -277.4874940834125141, -338.2021623163374215 ) ) ;
#81054=CARTESIAN_POINT ( 'NONE',  ( -112.3409153512424297, -286.5567344017749747, -270.0170808755260623 ) ) ;
#81058=CARTESIAN_POINT ( 'NONE',  ( -113.3892119865381574, -296.5375164170397966, -258.2038337485387842 ) ) ;
#81059=CARTESIAN_POINT ( 'NONE',  ( -6.356235243700066206, -288.4410580755821911, -202.4372341950638088 ) ) ;
#81061=CARTESIAN_POINT ( 'NONE',  ( -99.90806341382575795, -293.4094976428775681, -320.2154176792147382 ) ) ;
#81062=CARTESIAN_POINT ( 'NONE',  ( -110.2515050878268426, -277.7748034725568118, -246.4092066451927394 ) ) ;
#81063=CARTESIAN_POINT ( 'NONE',  ( -67.98812607131755215, -290.0563851197890699, -200.5813163142338738 ) ) ;
#81064=CARTESIAN_POINT ( 'NONE',  ( -71.51678181549092983, -287.1122146640895494, -205.0712141259976136 ) ) ;
#81065=CARTESIAN_POINT ( 'NONE',  ( -93.87857215656791254, -280.9819653218258395, -222.5759777706735463 ) ) ;
#81066=CARTESIAN_POINT ( 'NONE',  ( 38.50798064533656628, -289.0992827698227643, -280.0304756630850420 ) ) ;
#81067=CARTESIAN_POINT ( 'NONE',  ( 35.89886190683343870, -283.7596727216234740, -286.5110630639703686 ) ) ;
#81068=CARTESIAN_POINT ( 'NONE',  ( 23.51935042613633442, -276.3488882282474606, -317.5516931681427195 ) ) ;
#81069=CARTESIAN_POINT ( 'NONE',  ( -66.18552049367583834, -295.6928304350341818, -201.5143255293843367 ) ) ;
#81070=CARTESIAN_POINT ( 'NONE',  ( -94.96038012907692405, -279.0775225141174474, -219.2818881581052892 ) ) ;
#81071=CARTESIAN_POINT ( 'NONE',  ( -110.1933854105593014, -298.6709517194341856, -255.0044317975683157 ) ) ;
#81074=CARTESIAN_POINT ( 'NONE',  ( -20.25526795762937127, -276.7662352645559167, -195.3538533559490702 ) ) ;
#81075=CARTESIAN_POINT ( 'NONE',  ( 17.37568445726946820, -273.0598127527824772, -217.5600284599838403 ) ) ;
#81077=CARTESIAN_POINT ( 'NONE',  ( -93.98426742187328387, -278.7124853701401435, -224.2134418521454791 ) ) ;
#81078=CARTESIAN_POINT ( 'NONE',  ( 22.43879563562683899, -276.1120401272316940, -222.4414599991953594 ) ) ;
#81079=CARTESIAN_POINT ( 'NONE',  ( -5.563894817473393317, -281.7030332560919419, -340.2395216810197098 ) ) ;
#81080=CARTESIAN_POINT ( 'NONE',  ( -39.97180380360236285, -290.8456640728059028, -344.3779728523724089 ) ) ;
#81081=CARTESIAN_POINT ( 'NONE',  ( -75.45058760562159250, -299.0740573700583695, -204.1913127847192868 ) ) ;
#81082=CARTESIAN_POINT ( 'NONE',  ( -57.30112750002992783, -299.0053553423152835, -196.3491747455985035 ) ) ;
#81083=CARTESIAN_POINT ( 'NONE',  ( -63.46397673707561182, -293.7111094890969412, -200.2351235796422202 ) ) ;
#81084=CARTESIAN_POINT ( 'NONE',  ( 36.28474852576971443, -279.7251665690557161, -283.8183955616313483 ) ) ;
#81085=CARTESIAN_POINT ( 'NONE',  ( 36.95562760380333600, -283.4127182693125633, -265.7544611261768068 ) ) ;
#81086=CARTESIAN_POINT ( 'NONE',  ( -100.6627215264306727, -271.1058108246733127, -230.8352397431230543 ) ) ;
#81087=CARTESIAN_POINT ( 'NONE',  ( -83.38344493765916354, -285.2711118183223675, -331.1447497554304391 ) ) ;
#81088=CARTESIAN_POINT ( 'NONE',  ( 21.41301934707465904, -287.0852999203791001, -314.2239903163523422 ) ) ;
#81089=CARTESIAN_POINT ( 'NONE',  ( 46.50794016136936193, 11.67038243352686422, -331.8346843585704846 ) ) ;
#81091=CARTESIAN_POINT ( 'NONE',  ( -54.38796339852894590, -287.8415736881570410, -344.9005210889691853 ) ) ;
#81092=CARTESIAN_POINT ( 'NONE',  ( -75.88350115612369962, -289.2491505352648460, -332.3822197162926386 ) ) ;
#81094=CARTESIAN_POINT ( 'NONE',  ( -12.81562848708069247, -287.4433219292967010, -197.6977550056344342 ) ) ;
#81095=CARTESIAN_POINT ( 'NONE',  ( 21.49570089064525291, -275.2796840825200775, -227.1147571160295229 ) ) ;
#81097=CARTESIAN_POINT ( 'NONE',  ( 38.92029238707755923, -292.3646596883158963, -261.7742424161612576 ) ) ;
#81098=CARTESIAN_POINT ( 'NONE',  ( 25.02948034077640571, -282.8009855733371296, -315.3628977539175935 ) ) ;
#81099=CARTESIAN_POINT ( 'NONE',  ( 33.94673017477119004, -283.4199389111307141, -297.5763243271287593 ) ) ;
#81100=CARTESIAN_POINT ( 'NONE',  ( -33.05568014553059442, -283.3328630566061292, -347.2336945856786201 ) ) ;
#81101=CARTESIAN_POINT ( 'NONE',  ( 4.931943334121755562, -280.9745944060103398, -210.8209923937971553 ) ) ;
#81102=CARTESIAN_POINT ( 'NONE',  ( -92.08974858914540107, -293.4094976428775681, -313.9805196606274080 ) ) ;
#81103=CARTESIAN_POINT ( 'NONE',  ( 139.2571438113172633, 180.4774994735251994, -241.5552550638034859 ) ) ;
#81105=CARTESIAN_POINT ( 'NONE',  ( 36.65065063670046897, -277.4072407555393625, -259.0875783784314308 ) ) ;
#81106=CARTESIAN_POINT ( 'NONE',  ( 152.8849392923119410, 207.2903029783794011, -216.9541755379844403 ) ) ;
#81107=CARTESIAN_POINT ( 'NONE',  ( -49.96337633816796853, -297.2354167151027582, -198.3570489480232197 ) ) ;
#81108=CARTESIAN_POINT ( 'NONE',  ( 39.17517298197189035, -293.1666106410748966, -278.8942770213425888 ) ) ;
#81109=CARTESIAN_POINT ( 'NONE',  ( -46.80064229255074082, -155.6065870646474991, -361.5538532369118343 ) ) ;
#81110=CARTESIAN_POINT ( 'NONE',  ( -37.23604188324430453, -296.6281871560266836, -193.9496097253216078 ) ) ;
#81111=CARTESIAN_POINT ( 'NONE',  ( -53.60443062215115617, -287.6641699959375273, -342.3469777737124105 ) ) ;
#81112=CARTESIAN_POINT ( 'NONE',  ( -6.225953906302037488, -296.4993180164240130, -337.7604935021706183 ) ) ;
#81113=CARTESIAN_POINT ( 'NONE',  ( 23.93604853365003038, -288.3070496038653800, -229.6946232054161214 ) ) ;
#81115=CARTESIAN_POINT ( 'NONE',  ( 15.32598778891112978, -295.2707988202014349, -326.2085428286755473 ) ) ;
#81116=CARTESIAN_POINT ( 'NONE',  ( -110.4519534791522659, -285.0371887254378862, -270.9160186227093163 ) ) ;
#81117=CARTESIAN_POINT ( 'NONE',  ( -3.612408327879128134, -297.2605349072478020, -193.7649110999839763 ) ) ;
#81118=CARTESIAN_POINT ( 'NONE',  ( -4.682081716713339503, -293.2743500184636787, -200.8089207022684093 ) ) ;
#81119=CARTESIAN_POINT ( 'NONE',  ( 33.36249715357018886, -294.4327441453648930, -300.8345012732876853 ) ) ;
#81120=CARTESIAN_POINT ( 'NONE',  ( -34.85940900976114420, -292.2508812796249345, -197.4033340569970960 ) ) ;
#81123=CARTESIAN_POINT ( 'NONE',  ( -35.88208377262943571, -299.9306490915744234, -194.5958537802862338 ) ) ;
#81124=CARTESIAN_POINT ( 'NONE',  ( 7.017615659521933225, -273.4359129123248522, -207.8439515411113803 ) ) ;
#81126=CARTESIAN_POINT ( 'NONE',  ( -75.31129124947567277, -277.0520165697235484, -337.2777605563284169 ) ) ;
#81127=CARTESIAN_POINT ( 'NONE',  ( -40.52876287109086917, -296.4912599921035508, -196.7240627453659840 ) ) ;
#81128=CARTESIAN_POINT ( 'NONE',  ( -111.6278932407283691, -280.4086155239939444, -270.6663847939050811 ) ) ;
#81129=CARTESIAN_POINT ( 'NONE',  ( 34.78103651359941750, -273.9205020976803553, -287.9980050952301553 ) ) ;
#81130=CARTESIAN_POINT ( 'NONE',  ( -66.99375193943554052, -298.8597163750683308, -203.2065673810634507 ) ) ;
#81131=CARTESIAN_POINT ( 'NONE',  ( -91.30399596762678982, -274.2018672948210565, -220.8301371711825425 ) ) ;
#81132=CARTESIAN_POINT ( 'NONE',  ( -75.93760363468544483, -275.3046920651395908, -204.8455145941681508 ) ) ;
#81133=CARTESIAN_POINT ( 'NONE',  ( -18.92697745587564384, -272.3080288994905800, -197.2367124416590514 ) ) ;
#81134=CARTESIAN_POINT ( 'NONE',  ( -105.0532035735895278, -296.8350223503308598, -297.9118887351315834 ) ) ;
#81135=CARTESIAN_POINT ( 'NONE',  ( 23.84114592328646154, -291.5635845737907061, -229.4706023793314387 ) ) ;
#81137=CARTESIAN_POINT ( 'NONE',  ( 30.49177328673300380, -276.5153797471604662, -306.7799177930620544 ) ) ;
#81138=CARTESIAN_POINT ( 'NONE',  ( 33.83328632781571343, -275.5041863207380857, -254.0842228874323325 ) ) ;
#81139=CARTESIAN_POINT ( 'NONE',  ( -80.64519636445542972, -284.1634609480477707, -207.2249561492333783 ) ) ;
#81140=CARTESIAN_POINT ( 'NONE',  ( -111.5829074091532362, -298.7040071300628483, -258.5205138357268879 ) ) ;
#81142=CARTESIAN_POINT ( 'NONE',  ( -10.68162471579387507, -285.6061263622431170, -202.2164956722405122 ) ) ;
#81143=CARTESIAN_POINT ( 'NONE',  ( -87.12680032124481500, -281.7431171282759124, -326.7464627112561288 ) ) ;
#81144=CARTESIAN_POINT ( 'NONE',  ( -105.2094247737140336, -276.3989058013166868, -300.0183623878365893 ) ) ;
#81145=CARTESIAN_POINT ( 'NONE',  ( -41.91116146937901021, -275.6855488254684019, -343.8210415753244433 ) ) ;
#81146=CARTESIAN_POINT ( 'NONE',  ( -72.09033144272315496, -281.5928239206886019, -203.8823139526549824 ) ) ;
#81147=CARTESIAN_POINT ( 'NONE',  ( 25.60853230369290756, -276.2397171162194240, -232.5215005462403610 ) ) ;
#81149=CARTESIAN_POINT ( 'NONE',  ( -4.155900712283271403, -272.8822561361930070, -201.7527120644970751 ) ) ;
#81150=CARTESIAN_POINT ( 'NONE',  ( -101.8515968014017830, -281.0687960857908365, -231.6787520485760012 ) ) ;
#81152=CARTESIAN_POINT ( 'NONE',  ( -72.95631528853381553, -287.5045709336444588, -203.6629816887706568 ) ) ;
#81154=CARTESIAN_POINT ( 'NONE',  ( -84.15084003026952075, -287.6950971216859898, -329.0263352753115669 ) ) ;
#81155=CARTESIAN_POINT ( 'NONE',  ( 82.13289967990638729, -300.8078083816499770, -196.9362037238964547 ) ) ;
#81156=CARTESIAN_POINT ( 'NONE',  ( -94.98917991864817623, -271.8759651007783873, -224.7759059781753592 ) ) ;
#81157=CARTESIAN_POINT ( 'NONE',  ( -111.4777333574609344, -288.7530537491341533, -265.6337423474823822 ) ) ;
#81158=CARTESIAN_POINT ( 'NONE',  ( -98.31850732666445936, -258.1384851437703674, -325.6453615436536211 ) ) ;
#81160=CARTESIAN_POINT ( 'NONE',  ( 37.14389035191657484, -286.2419176999983392, -286.9919003115932696 ) ) ;
#81161=CARTESIAN_POINT ( 'NONE',  ( -38.88156114600245417, -284.6718822012624059, -344.1576822308709893 ) ) ;
#81162=CARTESIAN_POINT ( 'NONE',  ( -108.0768612491187639, -283.1502107414489728, -242.4600521636990322 ) ) ;
#81163=CARTESIAN_POINT ( 'NONE',  ( -104.7030699935923224, -290.9310985910718728, -242.0969267024317730 ) ) ;
#81164=CARTESIAN_POINT ( 'NONE',  ( 28.29883504831773422, -282.5280022861361999, -236.9811566978089559 ) ) ;
#81165=CARTESIAN_POINT ( 'NONE',  ( -8.421022560577354099, -283.4664089788720958, -337.5637677543663244 ) ) ;
#81166=CARTESIAN_POINT ( 'NONE',  ( -26.35883693561027385, -290.8929229774543614, -344.9116613525393973 ) ) ;
#81167=CARTESIAN_POINT ( 'NONE',  ( -48.97208509230587481, -298.0747154951972107, -194.1908688108873946 ) ) ;
#81168=CARTESIAN_POINT ( 'NONE',  ( -43.09745856201845982, -287.2041386406997958, -345.7015815009527273 ) ) ;
#81169=CARTESIAN_POINT ( 'NONE',  ( 35.20097124020939816, -275.8797668597750317, -296.3361183855998320 ) ) ;
#81170=CARTESIAN_POINT ( 'NONE',  ( -75.84926095790396516, -293.5156267409894326, -206.3553586539070750 ) ) ;
#81172=CARTESIAN_POINT ( 'NONE',  ( -37.37352853689063892, -282.5519495502701943, -195.3611179825600175 ) ) ;
#81173=CARTESIAN_POINT ( 'NONE',  ( -111.4251638451020625, -276.7148886522541034, -257.6462120927429851 ) ) ;
#81175=CARTESIAN_POINT ( 'NONE',  ( -100.0802968076212522, -295.5292642151891869, -227.0911278678306644 ) ) ;
#81176=CARTESIAN_POINT ( 'NONE',  ( -3.828115394928857995, -275.9463152518902689, -335.3282812792550658 ) ) ;
#81177=CARTESIAN_POINT ( 'NONE',  ( -110.9393000054353848, -292.1330474482526256, -265.7109778318026088 ) ) ;
#81178=CARTESIAN_POINT ( 'NONE',  ( -66.66927161994094320, -292.5995071177352429, -203.2544715230085330 ) ) ;
#81179=CARTESIAN_POINT ( 'NONE',  ( -89.59403115579823407, -285.5608774909879344, -322.8512329352829511 ) ) ;
#81180=CARTESIAN_POINT ( 'NONE',  ( 39.06610522908409422, -294.9406199826531179, -267.4408758182344172 ) ) ;
#81181=CARTESIAN_POINT ( 'NONE',  ( 32.86517394689387572, -294.4773977508162375, -239.9589288487968304 ) ) ;
#81182=CARTESIAN_POINT ( 'NONE',  ( 35.53482023703489290, -293.3189499881820552, -265.3184566903651103 ) ) ;
#81183=CARTESIAN_POINT ( 'NONE',  ( 37.26126986915375028, -289.4533585890311542, -262.6541396555891197 ) ) ;
#81184=CARTESIAN_POINT ( 'NONE',  ( 34.58826261581754835, -282.0667149979192345, -297.8398454667993178 ) ) ;
#81185=CARTESIAN_POINT ( 'NONE',  ( -112.9466463274225134, -270.7637583252351305, -264.6946417773449980 ) ) ;
#81186=CARTESIAN_POINT ( 'NONE',  ( -85.51125822836189627, -285.2400396894515779, -210.2887143606990605 ) ) ;
#81187=CARTESIAN_POINT ( 'NONE',  ( 18.68613221842540995, -278.2209581168903583, -319.7031097048322295 ) ) ;
#81188=CARTESIAN_POINT ( 'NONE',  ( -42.68782004208540570, -284.7781555897413455, -197.1463096205446845 ) ) ;
#81189=CARTESIAN_POINT ( 'NONE',  ( 26.99632535157911661, -285.0347991573499371, -231.7171722181275868 ) ) ;
#81190=CARTESIAN_POINT ( 'NONE',  ( -109.3679212725146215, -276.9941848409339968, -246.6888339108536456 ) ) ;
#81191=CARTESIAN_POINT ( 'NONE',  ( -114.4693268140674434, -273.6886850827510216, -284.2063049943780015 ) ) ;
#81192=CARTESIAN_POINT ( 'NONE',  ( -87.73241653717960276, -284.8324266291617732, -217.4577708169034622 ) ) ;
#81193=CARTESIAN_POINT ( 'NONE',  ( 36.59769847098299067, -282.5045859886839708, -250.2870757476581218 ) ) ;
#81194=CARTESIAN_POINT ( 'NONE',  ( -70.54817239863834288, -288.5380006093341194, -339.5864729170215810 ) ) ;
#81195=CARTESIAN_POINT ( 'NONE',  ( 34.93456752430741119, -295.1041237575412310, -254.3616042233055055 ) ) ;
#81196=CARTESIAN_POINT ( 'NONE',  ( -48.35797936653824536, -278.7901101711087790, -345.8139334309867650 ) ) ;
#81197=CARTESIAN_POINT ( 'NONE',  ( 16.61935737316933981, -277.6196551414937517, -324.6707318905287138 ) ) ;
#81198=CARTESIAN_POINT ( 'NONE',  ( -24.87430416598558480, -280.0489614866456805, -198.4336264204988254 ) ) ;
#81199=CARTESIAN_POINT ( 'NONE',  ( -35.10398325353420290, -300.0803836229325157, -195.5270108691089490 ) ) ;
#81200=CARTESIAN_POINT ( 'NONE',  ( 28.63509732596806501, -286.0228955493852823, -305.7855054670853292 ) ) ;
#81201=CARTESIAN_POINT ( 'NONE',  ( -110.0126609545595926, -291.8592385785266288, -293.4543401422267266 ) ) ;
#81202=CARTESIAN_POINT ( 'NONE',  ( -50.54029706534402067, -294.1450064490936143, -342.4723037419922775 ) ) ;
#81204=CARTESIAN_POINT ( 'NONE',  ( -39.69396982502791360, -294.7491881178716540, -343.3567987811692319 ) ) ;
#81205=CARTESIAN_POINT ( 'NONE',  ( -109.5697662326491724, -291.3033273372230951, -296.2982938339348493 ) ) ;
#81206=CARTESIAN_POINT ( 'NONE',  ( -98.08292487737951149, -279.7687812167593506, -229.5969493747275578 ) ) ;
#81208=CARTESIAN_POINT ( 'NONE',  ( -109.8756055228439834, -271.9287356430028240, -245.2284145694832489 ) ) ;
#81209=CARTESIAN_POINT ( 'NONE',  ( 24.06582193259179903, -288.8207150812963846, -316.6474984990423991 ) ) ;
#81210=CARTESIAN_POINT ( 'NONE',  ( -8.237192175341450096, -289.0146020207796482, -341.6401820037439734 ) ) ;
#81211=CARTESIAN_POINT ( 'NONE',  ( -93.27403225407111620, -285.5518670442850748, -223.4179426553355938 ) ) ;
#81213=CARTESIAN_POINT ( 'NONE',  ( 82.92025895306024097, 83.20676217455302037, -300.2504679712564553 ) ) ;
#81214=CARTESIAN_POINT ( 'NONE',  ( -70.26940817115894333, -195.8484599149890073, -356.6074167248179378 ) ) ;
#81215=CARTESIAN_POINT ( 'NONE',  ( 11.84872889966633736, -275.5452533590565167, -324.5861405847504102 ) ) ;
#81216=CARTESIAN_POINT ( 'NONE',  ( -103.6435683292885415, -277.8947443028860107, -238.9642479356203069 ) ) ;
#81217=CARTESIAN_POINT ( 'NONE',  ( -95.06780847111842547, -272.9086296281636805, -219.4352826223653494 ) ) ;
#81218=CARTESIAN_POINT ( 'NONE',  ( 104.4767245839417882, 114.1861031128568129, -280.3257878957174398 ) ) ;
#81219=CARTESIAN_POINT ( 'NONE',  ( -48.43911547166732134, -275.8752772437485419, -346.1123941580989367 ) ) ;
#81220=CARTESIAN_POINT ( 'NONE',  ( -71.59689116425990107, -297.2586104950106574, -338.1885158671365730 ) ) ;
#81221=CARTESIAN_POINT ( 'NONE',  ( -57.67807833190245503, -292.2748651219350222, -200.1339822480225337 ) ) ;
#81222=CARTESIAN_POINT ( 'NONE',  ( -95.45569687099602163, -298.0361162550571521, -220.0131935004228581 ) ) ;
#81223=CARTESIAN_POINT ( 'NONE',  ( -36.90359686735268241, -298.5498438543773432, -193.4226204581699164 ) ) ;
#81224=CARTESIAN_POINT ( 'NONE',  ( -70.46944551625000486, -297.7694525685462850, -205.2968219823161746 ) ) ;
#81227=CARTESIAN_POINT ( 'NONE',  ( -111.3776692228935161, -280.2790515053716263, -285.5242811224306365 ) ) ;
#81228=CARTESIAN_POINT ( 'NONE',  ( -41.57202976823054286, -282.6116064330056474, -347.2354775583726223 ) ) ;
#81229=CARTESIAN_POINT ( 'NONE',  ( -92.44985349180895184, -280.3191176864269210, -221.9962056982960803 ) ) ;
#81230=CARTESIAN_POINT ( 'NONE',  ( -108.7763599518977884, -279.9789757689379144, -296.4198064831964530 ) ) ;
#81231=CARTESIAN_POINT ( 'NONE',  ( -64.80940502125579883, -272.1666873750790501, -201.9645246539039363 ) ) ;
#81234=CARTESIAN_POINT ( 'NONE',  ( -27.56047655018827669, -280.3464107401491674, -197.9681849790304398 ) ) ;
#81235=CARTESIAN_POINT ( 'NONE',  ( 33.56059034655385176, -275.9760130332741142, -240.6091487538548961 ) ) ;
#81236=CARTESIAN_POINT ( 'NONE',  ( 36.25122665503943153, -277.3666505411950993, -255.9014575707936956 ) ) ;
#81237=CARTESIAN_POINT ( 'NONE',  ( -4.266453781182229399, -275.1994211951595162, -339.2568102565784898 ) ) ;
#81240=CARTESIAN_POINT ( 'NONE',  ( 12.60975930829918035, -284.3402093709125893, -326.8509687194577396 ) ) ;
#81241=CARTESIAN_POINT ( 'NONE',  ( -49.70597577007611534, -291.0877180726020583, -198.2005511889541367 ) ) ;
#81242=CARTESIAN_POINT ( 'NONE',  ( -63.15939255558951260, -285.0730949495654158, -197.9265989727552437 ) ) ;
#81243=CARTESIAN_POINT ( 'NONE',  ( -111.3328080770970274, -282.7490649166518324, -273.6612706559420758 ) ) ;
#81244=CARTESIAN_POINT ( 'NONE',  ( -8.278098004815507949, -281.2386641966512570, -337.9679367943122656 ) ) ;
#81245=CARTESIAN_POINT ( 'NONE',  ( 36.70932245555122364, -285.5336757920342166, -262.7611014771114810 ) ) ;
#81246=CARTESIAN_POINT ( 'NONE',  ( 2.908983637272627654, -281.8103999212079884, -208.9241445252194751 ) ) ;
#81247=CARTESIAN_POINT ( 'NONE',  ( -108.2036598348584988, -270.8699978517628892, -245.7931853405240759 ) ) ;
#81248=CARTESIAN_POINT ( 'NONE',  ( -61.00282083519147847, -281.7539872453096450, -342.8495905510337707 ) ) ;
#81249=CARTESIAN_POINT ( 'NONE',  ( 35.80491741264854255, -295.3388831302748940, -253.7333811615970944 ) ) ;
#81250=CARTESIAN_POINT ( 'NONE',  ( -87.15894502997495863, -278.4200999510301244, -323.8600411337701530 ) ) ;
#81251=CARTESIAN_POINT ( 'NONE',  ( -49.08406813156094017, -287.9031698753166779, -196.0648369469861905 ) ) ;
#81255=CARTESIAN_POINT ( 'NONE',  ( -101.9965865210954377, -292.9935195910395578, -231.1569917194355241 ) ) ;
#81256=CARTESIAN_POINT ( 'NONE',  ( 36.60166337140330484, -273.3899329055136604, -257.7395825494043038 ) ) ;
#81257=CARTESIAN_POINT ( 'NONE',  ( -75.59218773248352363, -288.7462402929367613, -337.0023891180822488 ) ) ;
#81258=CARTESIAN_POINT ( 'NONE',  ( 28.20632927188960082, -291.4958893708869141, -236.4509977397852651 ) ) ;
#81260=CARTESIAN_POINT ( 'NONE',  ( -99.60172158447142010, -276.7002309264416908, -309.5066041128490610 ) ) ;
#81261=CARTESIAN_POINT ( 'NONE',  ( -108.0529894272545732, -294.3950627734656678, -293.1281215358523013 ) ) ;
#81262=CARTESIAN_POINT ( 'NONE',  ( -109.7656357839777570, -292.0348096266854441, -257.5795006073743707 ) ) ;
#81265=CARTESIAN_POINT ( 'NONE',  ( 3.784309863321918321, -291.0744258250283565, -206.0228280620011674 ) ) ;
#81266=CARTESIAN_POINT ( 'NONE',  ( 28.36118508618228518, -288.6992533750243979, -236.6394093944941233 ) ) ;
#81267=CARTESIAN_POINT ( 'NONE',  ( -87.95758496441295904, -289.5954569490654649, -213.6865539008864232 ) ) ;
#81268=CARTESIAN_POINT ( 'NONE',  ( -8.036849414009644477, -287.8690213044634447, -202.8585206774452274 ) ) ;
#81270=CARTESIAN_POINT ( 'NONE',  ( 35.12172837380102663, -288.4888993508541262, -280.5347457627498784 ) ) ;
#81271=CARTESIAN_POINT ( 'NONE',  ( 24.38219372006125596, -296.1163363189299389, -313.6105805481400921 ) ) ;
#81273=CARTESIAN_POINT ( 'NONE',  ( -34.66524695905027897, -290.2242894414718535, -346.9172759190810780 ) ) ;
#81274=CARTESIAN_POINT ( 'NONE',  ( -89.89266497888856122, -277.3352484817424966, -216.2809644601839523 ) ) ;
#81275=CARTESIAN_POINT ( 'NONE',  ( -59.65482564042597602, -277.6667666883224115, -344.0351888713203721 ) ) ;
#81276=CARTESIAN_POINT ( 'NONE',  ( 21.05283429031712217, -280.5414857760982841, -220.1830962588607292 ) ) ;
#81277=CARTESIAN_POINT ( 'NONE',  ( -111.0114230219513161, -274.6150527521714935, -259.3269491315330697 ) ) ;
#81278=CARTESIAN_POINT ( 'NONE',  ( -98.98564862407852161, -283.1316085372211546, -227.6181247792901843 ) ) ;
#81280=CARTESIAN_POINT ( 'NONE',  ( -62.70914154084307768, -277.8581682846553917, -200.5404094773799102 ) ) ;
#81281=CARTESIAN_POINT ( 'NONE',  ( -105.2070147809307770, -282.1321585583525575, -302.2875915225437780 ) ) ;
#81282=CARTESIAN_POINT ( 'NONE',  ( -109.4300603157634129, -269.0111957867250112, -295.3470538382887867 ) ) ;
#81283=CARTESIAN_POINT ( 'NONE',  ( -62.19860101427708088, -275.8493931374848671, -342.5615171215882242 ) ) ;
#81284=CARTESIAN_POINT ( 'NONE',  ( -109.9623686681617301, -298.2359860622638053, -257.8332987720730216 ) ) ;
#81285=CARTESIAN_POINT ( 'NONE',  ( -113.5979705919323379, -283.3701060021716103, -278.5142599687440566 ) ) ;
#81286=CARTESIAN_POINT ( 'NONE',  ( -55.36312153228242749, -298.7559470015147554, -199.3252804010661805 ) ) ;
#81287=CARTESIAN_POINT ( 'NONE',  ( -97.36159442831041133, -274.6147419195990551, -223.0724450925362135 ) ) ;
#81288=CARTESIAN_POINT ( 'NONE',  ( 0.6270834835491304604, -274.2403444553486906, -207.9875742495381701 ) ) ;
#81289=CARTESIAN_POINT ( 'NONE',  ( -3.965314640643761379, -294.4924206900255967, -203.1827047360903293 ) ) ;
#81290=CARTESIAN_POINT ( 'NONE',  ( -93.59134379385628222, -290.0010702836752330, -323.0210130841915657 ) ) ;
#81291=CARTESIAN_POINT ( 'NONE',  ( -53.42958015600600419, -277.9273395718526558, -196.4801097755100727 ) ) ;
#81292=CARTESIAN_POINT ( 'NONE',  ( -96.39242224725961705, -289.7202298037295805, -319.7982899446544138 ) ) ;
#81293=CARTESIAN_POINT ( 'NONE',  ( -68.87009993124429741, -288.5359539375419899, -336.4623165707907333 ) ) ;
#81294=CARTESIAN_POINT ( 'NONE',  ( 33.57020032810189036, -291.2341105417483504, -245.7803418904064472 ) ) ;
#81297=CARTESIAN_POINT ( 'NONE',  ( -94.33497372814193227, -290.7055407066397947, -224.6273991964368975 ) ) ;
#81299=CARTESIAN_POINT ( 'NONE',  ( 31.20628789008248205, -288.0473889107122432, -235.8069062139917662 ) ) ;
#81300=CARTESIAN_POINT ( 'NONE',  ( -53.28691492658256834, -285.7662352645559736, -340.3683826091709079 ) ) ;
#81301=CARTESIAN_POINT ( 'NONE',  ( 32.01228332807568222, -293.0353065566533246, -303.3916041617171686 ) ) ;
#81302=CARTESIAN_POINT ( 'NONE',  ( -30.24386454247041911, -284.2792983634745951, -346.5380108207003218 ) ) ;
#81303=CARTESIAN_POINT ( 'NONE',  ( -109.4986889700974189, -284.2352655521664815, -281.7475375758394307 ) ) ;
#81304=CARTESIAN_POINT ( 'NONE',  ( 28.47958570605879558, -277.3090026658273928, -303.1684304172225666 ) ) ;
#81305=CARTESIAN_POINT ( 'NONE',  ( -34.77605330411625317, -290.1046560923730908, -195.7604191807333791 ) ) ;
#81306=CARTESIAN_POINT ( 'NONE',  ( 15.74453713689562662, -273.6192544356102303, -219.6024046098876283 ) ) ;
#81308=LINE ( 'NONE', #74211, #80348 ) ;
#81309=CARTESIAN_POINT ( 'NONE',  ( -37.30422292179076038, -287.9727411305697728, -195.9084390689546353 ) ) ;
#81310=CARTESIAN_POINT ( 'NONE',  ( -113.3443784492282020, -297.4982220499722985, -281.0006568820179496 ) ) ;
#81311=CARTESIAN_POINT ( 'NONE',  ( -44.04196611058176103, -286.6166151926872203, -197.5668935966541540 ) ) ;
#81312=CARTESIAN_POINT ( 'NONE',  ( -113.4821331940253089, -277.7385326713653626, -260.1871278906868383 ) ) ;
#81313=CARTESIAN_POINT ( 'NONE',  ( 35.35352747067980772, -293.8852568680878790, -245.1257620952529521 ) ) ;
#81314=CARTESIAN_POINT ( 'NONE',  ( 26.39269665070026605, -286.2390620322331074, -311.4240389712932711 ) ) ;
#81315=CARTESIAN_POINT ( 'NONE',  ( 38.58613285433296625, -294.0450194006032802, -283.1180974408335942 ) ) ;
#81316=CARTESIAN_POINT ( 'NONE',  ( -70.23404068746381768, -291.9394870254791954, -205.1677025221914334 ) ) ;
#81318=CARTESIAN_POINT ( 'NONE',  ( 85.09997405915690649, 81.31097194785500903, -298.9058856463690290 ) ) ;
#81319=CARTESIAN_POINT ( 'NONE',  ( -80.56158883095672252, -286.9983004016568771, -207.4105338568816137 ) ) ;
#81320=CARTESIAN_POINT ( 'NONE',  ( -72.02372285203398405, -277.1237833571632905, -198.2697987213421698 ) ) ;
#81322=CARTESIAN_POINT ( 'NONE',  ( -18.67012212205499111, -281.7264401183609266, -341.3051949448220626 ) ) ;
#81323=CARTESIAN_POINT ( 'NONE',  ( -104.7730214049796871, -278.6999484682532398, -233.2294441407206875 ) ) ;
#81324=CARTESIAN_POINT ( 'NONE',  ( 36.03320654325722927, -283.7423361360032459, -285.1278041019679677 ) ) ;
#81325=CARTESIAN_POINT ( 'NONE',  ( 66.82556401647084954, 46.20335925335534455, -317.4906725690062785 ) ) ;
#81326=CARTESIAN_POINT ( 'NONE',  ( -58.34236709178786384, -281.8930107278820856, -343.8844082265167685 ) ) ;
#81327=CARTESIAN_POINT ( 'NONE',  ( 23.34318196787115696, -284.9771508198932111, -226.8091009963864337 ) ) ;
#81328=CARTESIAN_POINT ( 'NONE',  ( -16.14599672560019528, -276.1836196671497987, -197.5670846912198328 ) ) ;
#81329=CARTESIAN_POINT ( 'NONE',  ( -71.69947979957566986, -298.0775888007794947, -205.8679853551003021 ) ) ;
#81330=CARTESIAN_POINT ( 'NONE',  ( -37.01003171226221156, -293.7327053368494489, -343.8660299603760109 ) ) ;
#81331=CARTESIAN_POINT ( 'NONE',  ( -106.0881764365554716, -279.6487025778943689, -235.7862254908652915 ) ) ;
#81332=CARTESIAN_POINT ( 'NONE',  ( -9.988363180829333388, -276.6847911203981312, -338.0562539702432332 ) ) ;
#81333=CARTESIAN_POINT ( 'NONE',  ( 30.51773547607830395, -299.8235251788059941, -193.5858418448398481 ) ) ;
#81334=CARTESIAN_POINT ( 'NONE',  ( 5.686445206171891975, -275.4042148266325967, -333.8439599020867377 ) ) ;
#81336=CARTESIAN_POINT ( 'NONE',  ( 26.82474003563958931, -274.0734160259896157, -309.2887839668493939 ) ) ;
#81337=CARTESIAN_POINT ( 'NONE',  ( -101.8289202621643312, -298.5187736273210817, -229.3732571988008715 ) ) ;
#81339=CARTESIAN_POINT ( 'NONE',  ( -110.2140734402150315, -271.0703965937372004, -283.6296548450457635 ) ) ;
#81340=CARTESIAN_POINT ( 'NONE',  ( -108.9698682338513009, -285.8376328758349700, -254.6937588525607907 ) ) ;
#81341=CARTESIAN_POINT ( 'NONE',  ( -52.69072012957874307, -285.0062027726391420, -344.8351931436837958 ) ) ;
#81342=CARTESIAN_POINT ( 'NONE',  ( 16.05458418754304262, -286.1833120211005621, -220.4154012836551999 ) ) ;
#81343=CARTESIAN_POINT ( 'NONE',  ( -83.52307047194003076, -276.0971419712317356, -327.9918357338194710 ) ) ;
#81344=CARTESIAN_POINT ( 'NONE',  ( -68.27787930424383944, -285.3233100589075093, -337.8431029952679410 ) ) ;
#81345=CARTESIAN_POINT ( 'NONE',  ( -93.60715118031951931, -277.7022325903813567, -222.7506770376182885 ) ) ;
#81346=CARTESIAN_POINT ( 'NONE',  ( 9.873583870998631440, -277.4633677864011361, -326.4409096151675271 ) ) ;
#81348=CARTESIAN_POINT ( 'NONE',  ( -46.19244642374174248, -274.4291911342560866, -197.8376546648480314 ) ) ;
#81349=CARTESIAN_POINT ( 'NONE',  ( 21.83978537285823762, -281.6947813910225022, -221.3538675489834588 ) ) ;
#81350=CARTESIAN_POINT ( 'NONE',  ( -53.75347074004272230, -280.3394526330582721, -195.1389079685595505 ) ) ;
#81354=CARTESIAN_POINT ( 'NONE',  ( 37.86747419535247161, -289.5343562493065974, -279.9430820895992724 ) ) ;
#81355=CARTESIAN_POINT ( 'NONE',  ( -109.2023493307237914, -295.9309814179370051, -256.5594944881757442 ) ) ;
#81356=CARTESIAN_POINT ( 'NONE',  ( -64.34522807906411401, -291.0575650914665289, -198.3041729302228475 ) ) ;
#81357=CARTESIAN_POINT ( 'NONE',  ( 33.74561369506310626, -286.2884649720591028, -289.9745456191522521 ) ) ;
#81358=CARTESIAN_POINT ( 'NONE',  ( 19.96097293214453572, -286.7744640986632021, -316.5323057434561065 ) ) ;
#81360=CARTESIAN_POINT ( 'NONE',  ( -94.44057324830791345, -286.4060842098854209, -224.2234177018688115 ) ) ;
#81361=CARTESIAN_POINT ( 'NONE',  ( -111.0263549127709410, -276.7324355071842206, -256.3078387516918610 ) ) ;
#81362=CARTESIAN_POINT ( 'NONE',  ( -20.69126801014350647, -287.2418510029499998, -344.7738281839484671 ) ) ;
#81363=CARTESIAN_POINT ( 'NONE',  ( -10.72811651100436059, -288.3992486793349030, -200.1864893045815847 ) ) ;
#81364=CARTESIAN_POINT ( 'NONE',  ( -72.34331628848264018, -287.5139770990570014, -336.8955619537001667 ) ) ;
#81365=CARTESIAN_POINT ( 'NONE',  ( 3.531447220981597468, -283.4290639767513653, -331.1908326551225628 ) ) ;
#81366=CARTESIAN_POINT ( 'NONE',  ( -111.8523868708366251, -292.6841544289595163, -260.0702160009950603 ) ) ;
#81367=CARTESIAN_POINT ( 'NONE',  ( 82.17440492340898572, -297.5479941798179766, -195.4018648718562758 ) ) ;
#81370=CARTESIAN_POINT ( 'NONE',  ( -43.20291855017449478, -299.8989806329308294, -194.9765699901674907 ) ) ;
#81371=CARTESIAN_POINT ( 'NONE',  ( -5.478949716187477392, -279.6795877892465114, -204.5024293851987238 ) ) ;
#81372=CARTESIAN_POINT ( 'NONE',  ( 36.67329314420914699, -279.7075511315860581, -282.4764562279408437 ) ) ;
#81373=CARTESIAN_POINT ( 'NONE',  ( -36.28694200525179525, -294.2364525765680696, -347.2054790667232282 ) ) ;
#81374=CARTESIAN_POINT ( 'NONE',  ( -98.67045888005063148, -271.3611402587774819, -228.8359544951688349 ) ) ;
#81375=CARTESIAN_POINT ( 'NONE',  ( 36.78577978026066830, -273.7201423301747809, -277.1751416586939740 ) ) ;
#81376=CARTESIAN_POINT ( 'NONE',  ( -10.29302344350573684, -296.0067533491657628, -338.6956814769762332 ) ) ;
#81378=CARTESIAN_POINT ( 'NONE',  ( -26.31477977795560008, -296.6677219392449274, -194.0572370515587295 ) ) ;
#81379=CARTESIAN_POINT ( 'NONE',  ( -78.94119356547467703, -293.8446010281147096, -333.9492942262800170 ) ) ;
#81380=CARTESIAN_POINT ( 'NONE',  ( 25.34032596684660632, -294.4490716688201246, -231.7113560091423210 ) ) ;
#81382=CARTESIAN_POINT ( 'NONE',  ( 27.62524867361743830, -293.8984636010243889, -236.7174367059492965 ) ) ;
#81383=CYLINDRICAL_SURFACE ( 'NONE', #74691, 6.654241149514406040 ) ;
#81384=CARTESIAN_POINT ( 'NONE',  ( -112.1830620587764145, -282.6845268662134458, -261.5760541710594111 ) ) ;
#81385=CARTESIAN_POINT ( 'NONE',  ( -50.47120694303523436, -295.2245040643452967, -342.1706998696318465 ) ) ;
#81386=CARTESIAN_POINT ( 'NONE',  ( 19.78351099337463026, -282.2539338830199540, -322.0696422999189963 ) ) ;
#81387=CARTESIAN_POINT ( 'NONE',  ( 7.668760580706223351, -282.5808814582451305, -209.6052980017566369 ) ) ;
#81388=CARTESIAN_POINT ( 'NONE',  ( -69.78006142819397439, -285.3033658619228277, -200.5363206065779877 ) ) ;
#81389=CARTESIAN_POINT ( 'NONE',  ( -78.23625058208033067, -289.5005245633677760, -207.6900387831504418 ) ) ;
#81391=CARTESIAN_POINT ( 'NONE',  ( -1.934187046497397588, -285.2159557426453489, -205.9025260038430076 ) ) ;
#81392=CARTESIAN_POINT ( 'NONE',  ( -96.16285584303419398, -288.8073861016825958, -319.5908826408016807 ) ) ;
#81394=CARTESIAN_POINT ( 'NONE',  ( -7.647927608291255730, -296.2564634006638471, -337.9375599932996579 ) ) ;
#81395=CARTESIAN_POINT ( 'NONE',  ( -112.7149367621744318, -279.8192653164257990, -282.9102810096326266 ) ) ;
#81396=CARTESIAN_POINT ( 'NONE',  ( 16.37106635171574354, -292.3144476596136201, -323.2874188217909364 ) ) ;
#81397=CARTESIAN_POINT ( 'NONE',  ( 32.97866413002670782, -281.4788522812967244, -290.0368354391640082 ) ) ;
#81398=CARTESIAN_POINT ( 'NONE',  ( -8.386067436567360645, -294.8502094787792771, -341.7658402314601176 ) ) ;
#81399=CARTESIAN_POINT ( 'NONE',  ( -110.1113746663502582, -282.3722212337845576, -290.7053718961213917 ) ) ;
#81400=CARTESIAN_POINT ( 'NONE',  ( -71.89597354845865596, -279.5090360629486668, -336.9412160895406032 ) ) ;
#81401=CARTESIAN_POINT ( 'NONE',  ( 6.193218587319894830, -293.5038060208798356, -329.3150502127592745 ) ) ;
#81402=CARTESIAN_POINT ( 'NONE',  ( -29.30121614929279161, -296.1526455479262268, -195.3638505560702470 ) ) ;
#81405=CARTESIAN_POINT ( 'NONE',  ( 25.52912028483387630, -284.0775065495608942, -310.6943117138903858 ) ) ;
#81406=CARTESIAN_POINT ( 'NONE',  ( -108.0307092747496966, -295.8155947024000056, -288.8782039335736158 ) ) ;
#81408=CARTESIAN_POINT ( 'NONE',  ( 31.95455697924147032, -279.4809262143061233, -303.7686719486574702 ) ) ;
#81409=CARTESIAN_POINT ( 'NONE',  ( -21.37833918266614930, -273.4490437758136068, -195.1990934799911770 ) ) ;
#81410=CARTESIAN_POINT ( 'NONE',  ( 33.59144544411675071, -289.2352063861476950, -299.1691354513337160 ) ) ;
#81411=CARTESIAN_POINT ( 'NONE',  ( -106.5706182956691492, -290.6930563875704365, -247.2017377264558888 ) ) ;
#81412=CARTESIAN_POINT ( 'NONE',  ( -65.09501091746756174, -281.2029266097997606, -202.0935452020635239 ) ) ;
#81413=CARTESIAN_POINT ( 'NONE',  ( -35.38936557030753249, -275.6771580834642350, -196.5743010034133249 ) ) ;
#81414=CARTESIAN_POINT ( 'NONE',  ( -6.589118888062201584, -279.2601040915910175, -203.7034982912537657 ) ) ;
#81415=CARTESIAN_POINT ( 'NONE',  ( -6.666977479457773192, -278.6495834704358572, -338.8013257726720440 ) ) ;
#81416=VERTEX_POINT ( 'NONE', #65390 ) ;
#81417=CARTESIAN_POINT ( 'NONE',  ( -96.93472160949181671, -273.0403422845866999, -221.5791674555806878 ) ) ;
#81418=CARTESIAN_POINT ( 'NONE',  ( 9.741089117532043318, -294.6257718584731720, -212.6355812249413191 ) ) ;
#81419=CARTESIAN_POINT ( 'NONE',  ( 128.9467878515196162, -293.3047352414760667, -195.3611179825600175 ) ) ;
#81421=CARTESIAN_POINT ( 'NONE',  ( -3.845742125410460233, -290.6288506239876028, -202.3885421346880946 ) ) ;
#81422=VECTOR ( 'NONE', #84057, 1000.000000000000000 ) ;
#81423=CARTESIAN_POINT ( 'NONE',  ( -109.1890653965824640, -272.2382006614454895, -256.8262100058338433 ) ) ;
#81425=CARTESIAN_POINT ( 'NONE',  ( -99.29592239190790792, -291.4761780387928525, -314.9299009550358619 ) ) ;
#81426=CARTESIAN_POINT ( 'NONE',  ( -69.85430415644619018, -285.9805209788416391, -337.9475929042657754 ) ) ;
#81427=CARTESIAN_POINT ( 'NONE',  ( 12.33246085699259709, -288.7453289605854820, -214.3227204541045694 ) ) ;
#81428=CARTESIAN_POINT ( 'NONE',  ( -4.278437262528261620, -274.6152354769872659, -337.5084252735588279 ) ) ;
#81429=CARTESIAN_POINT ( 'NONE',  ( -1.041374552024579847, -276.4580071578250227, -205.3572902395208075 ) ) ;
#81430=CARTESIAN_POINT ( 'NONE',  ( -75.70109231751027323, -289.6162094113578291, -206.5054070283297563 ) ) ;
#81431=CARTESIAN_POINT ( 'NONE',  ( -83.82805160294078917, -281.2824061446086148, -210.4672535462808014 ) ) ;
#81434=CARTESIAN_POINT ( 'NONE',  ( -2.387209970727946384, -281.9253189169133407, -334.5788242504833647 ) ) ;
#81435=CARTESIAN_POINT ( 'NONE',  ( -111.4359621981392507, -279.8811430163831915, -250.5231947129944956 ) ) ;
#81437=CARTESIAN_POINT ( 'NONE',  ( -5.633954510387108705, -281.4392521888790384, -340.0936612302977551 ) ) ;
#81438=CARTESIAN_POINT ( 'NONE',  ( 5.749137854813886506, -277.4248127276291598, -333.8906378482966488 ) ) ;
#81440=CARTESIAN_POINT ( 'NONE',  ( 38.45129827353991203, -277.1894236963454432, -279.6441618940204989 ) ) ;
#81441=CARTESIAN_POINT ( 'NONE',  ( -6.941161984400275209, -291.1233781216987495, -333.4151289067050357 ) ) ;
#81444=CARTESIAN_POINT ( 'NONE',  ( -107.8591793374336589, -298.2193793707130567, -296.0535669861957899 ) ) ;
#81445=CARTESIAN_POINT ( 'NONE',  ( -15.74752801627614396, -289.8459273966242904, -340.4707034162061063 ) ) ;
#81446=CARTESIAN_POINT ( 'NONE',  ( -24.06118893897670574, -274.9019504825189415, -343.8676214626292449 ) ) ;
#81447=CARTESIAN_POINT ( 'NONE',  ( -2.248520732216863660, -290.3542664703600167, -337.7587646469406195 ) ) ;
#81448=CARTESIAN_POINT ( 'NONE',  ( -57.67534972201610799, -291.1312888155581504, -200.0911101867267234 ) ) ;
#81449=CARTESIAN_POINT ( 'NONE',  ( 39.02868673217405160, -287.1819724656100448, -280.1216023615793347 ) ) ;
#81451=CARTESIAN_POINT ( 'NONE',  ( -66.89848307319547871, -281.8459238038355466, -337.9975948380028399 ) ) ;
#81452=CARTESIAN_POINT ( 'NONE',  ( -81.11709823628069671, -291.5139719558001161, -330.3798859420436429 ) ) ;
#81453=CARTESIAN_POINT ( 'NONE',  ( -109.0355722145596928, -283.2554844095222393, -253.2570102271590144 ) ) ;
#81454=CARTESIAN_POINT ( 'NONE',  ( 34.13366569337756573, -283.0921338086079686, -287.5177939692293307 ) ) ;
#81455=CARTESIAN_POINT ( 'NONE',  ( 18.48196404994004993, -289.2151711512897805, -323.0539897076217812 ) ) ;
#81456=CARTESIAN_POINT ( 'NONE',  ( -100.6330112341380953, -278.5432377405155648, -306.9620047640015059 ) ) ;
#81457=CARTESIAN_POINT ( 'NONE',  ( -68.15489172491606951, -290.4513739081874064, -200.2144094642738708 ) ) ;
#81458=CARTESIAN_POINT ( 'NONE',  ( -43.66319970291937835, -286.7771650855093526, -193.7299220376817743 ) ) ;
#81459=CARTESIAN_POINT ( 'NONE',  ( 39.57839156035623063, -288.0234559837098232, -268.6799286120365764 ) ) ;
#81460=CARTESIAN_POINT ( 'NONE',  ( -107.7605909859749431, -284.4640800756865815, -289.6483647304665396 ) ) ;
#81463=CARTESIAN_POINT ( 'NONE',  ( -61.32048074744731281, -293.6045735923605093, -198.4356701956213556 ) ) ;
#81464=CARTESIAN_POINT ( 'NONE',  ( 37.28402649504832311, -292.0240855542635927, -253.4411470878083037 ) ) ;
#81465=CARTESIAN_POINT ( 'NONE',  ( -78.77496429265643485, -276.6841147795372535, -330.8107311738360181 ) ) ;
#81467=CARTESIAN_POINT ( 'NONE',  ( -51.77333915807633957, -297.2208882694891372, -194.7751326927263165 ) ) ;
#81468=CARTESIAN_POINT ( 'NONE',  ( 33.41046195464509339, -292.3026504975281910, -291.0180623975079470 ) ) ;
#81469=CARTESIAN_POINT ( 'NONE',  ( -105.9089854201567675, -294.4238561900944546, -298.2268926734060415 ) ) ;
#81470=CARTESIAN_POINT ( 'NONE',  ( -105.0754000392019947, -292.1359803686528380, -241.9573154962923525 ) ) ;
#81471=CARTESIAN_POINT ( 'NONE',  ( 35.95157311956521085, -294.6729113895875685, -273.4885028503704234 ) ) ;
#81472=FACE_OUTER_BOUND ( 'NONE', #85546, .T. ) ;
#81473=CARTESIAN_POINT ( 'NONE',  ( -39.09132017121444846, -293.0739058119107199, -345.5074236786803681 ) ) ;
#81474=CARTESIAN_POINT ( 'NONE',  ( -75.36370812783209772, -299.5457771993484926, -205.6547606666991896 ) ) ;
#81475=CARTESIAN_POINT ( 'NONE',  ( 32.54174415005469001, -288.7847564620081471, -292.4323337025993510 ) ) ;
#81476=CARTESIAN_POINT ( 'NONE',  ( 35.30677965448295907, -277.7888002471546542, -290.4244152352820265 ) ) ;
#81477=CARTESIAN_POINT ( 'NONE',  ( -88.58862666975814193, -278.0356210561185435, -213.5539811804669910 ) ) ;
#81478=CARTESIAN_POINT ( 'NONE',  ( -1.341860430457181064, -273.8655115880363837, -202.4102215307920289 ) ) ;
#81479=CARTESIAN_POINT ( 'NONE',  ( 36.46376833751075708, -279.5015557598004534, -260.2781165315608405 ) ) ;
#81480=CARTESIAN_POINT ( 'NONE',  ( -73.73291075551577478, -275.9268137223404551, -337.3246045073453274 ) ) ;
#81482=CARTESIAN_POINT ( 'NONE',  ( -95.17179299640066859, -294.6017628289737900, -315.7144402254459123 ) ) ;
#81483=CARTESIAN_POINT ( 'NONE',  ( -64.71025148262748417, -275.6949772249146235, -200.5193411917497031 ) ) ;
#81484=CARTESIAN_POINT ( 'NONE',  ( -78.91985458104686302, -274.1268321491026541, -210.1735099633457651 ) ) ;
#81485=AXIS2_PLACEMENT_3D ( 'NONE', #10114, #38980, #67893 ) ;
#81487=CARTESIAN_POINT ( 'NONE',  ( -95.29734249440812732, -289.2342558586020687, -222.1794760285708037 ) ) ;
#81488=CARTESIAN_POINT ( 'NONE',  ( -114.3688399610460635, -290.5772450426365481, -268.3547120787731046 ) ) ;
#81489=CARTESIAN_POINT ( 'NONE',  ( -93.72847377785052458, -275.2416943149733584, -220.6563879686030702 ) ) ;
#81490=CARTESIAN_POINT ( 'NONE',  ( -107.7198665985480233, -294.2197028883838925, -295.9486879867826019 ) ) ;
#81491=CARTESIAN_POINT ( 'NONE',  ( -58.45222210322820899, -282.5153502516368462, -344.2981959699600907 ) ) ;
#81493=CARTESIAN_POINT ( 'NONE',  ( -67.50851954882334383, -281.4476789634111924, -339.0405383877470058 ) ) ;
#81494=CARTESIAN_POINT ( 'NONE',  ( 129.4467878515196162, -299.5541904835127980, -195.3611179825600175 ) ) ;
#81495=CARTESIAN_POINT ( 'NONE',  ( -109.0955318707426898, -289.5497042579262370, -254.9170855964073041 ) ) ;
#81496=CARTESIAN_POINT ( 'NONE',  ( -89.78336789831863030, -281.9409037893129835, -322.9760100402969556 ) ) ;
#81497=DIRECTION ( 'NONE',  ( 0.000000000000000000, 0.000000000000000000, 1.000000000000000000 ) ) ;
#81499=CARTESIAN_POINT ( 'NONE',  ( 33.41874587569338217, -291.8757249217769072, -295.3752671500746487 ) ) ;
#81500=CARTESIAN_POINT ( 'NONE',  ( -87.62589355168771021, -279.3686623335170225, -324.3790807862029624 ) ) ;
#81501=CARTESIAN_POINT ( 'NONE',  ( -104.0635800021767494, -285.2651340506965312, -308.1009423208942053 ) ) ;
#81502=CARTESIAN_POINT ( 'NONE',  ( -49.46366225083603752, -271.9787532176643481, -195.7270078547863648 ) ) ;
#81503=CARTESIAN_POINT ( 'NONE',  ( -33.23865699473719104, -286.1051135741359985, -197.4266971368483894 ) ) ;
#81504=CARTESIAN_POINT ( 'NONE',  ( -3.581105182315538205, -278.0226648926341113, -335.7491684772039093 ) ) ;
#81505=CARTESIAN_POINT ( 'NONE',  ( -37.80053278590420263, -277.8608422846659778, -343.5336368507983025 ) ) ;
#81506=CARTESIAN_POINT ( 'NONE',  ( -100.8391223664173850, -287.0888725477194043, -230.4477365575937426 ) ) ;
#81509=CARTESIAN_POINT ( 'NONE',  ( -74.60822251473014433, -295.3668414701115807, -337.8018845265034997 ) ) ;
#81510=CARTESIAN_POINT ( 'NONE',  ( -44.20004833608461325, -287.9448798957060944, -196.0320532614270803 ) ) ;
#81512=CARTESIAN_POINT ( 'NONE',  ( -115.3288506153726871, -294.2666405000204009, -252.5284128619063608 ) ) ;
#81513=CARTESIAN_POINT ( 'NONE',  ( -113.7346718246339208, -277.5645414789357801, -263.0297439466132232 ) ) ;
#81514=CARTESIAN_POINT ( 'NONE',  ( -66.68831987432899666, -290.0739243870403925, -200.0388858949283986 ) ) ;
#81515=CARTESIAN_POINT ( 'NONE',  ( -98.69492629326609290, -286.6336142422166517, -229.5384601609094659 ) ) ;
#81516=CARTESIAN_POINT ( 'NONE',  ( -81.91577897981534306, -281.1958574203101193, -211.2110024554951337 ) ) ;
#81517=CARTESIAN_POINT ( 'NONE',  ( -52.07756747361237615, -287.2924948895428656, -195.3307418806546423 ) ) ;
#81518=CARTESIAN_POINT ( 'NONE',  ( 24.24114958020114230, -284.1330263699405805, -313.1694497831790613 ) ) ;
#81519=CARTESIAN_POINT ( 'NONE',  ( 37.90613039848756216, -275.9238673877632664, -286.7556407575713706 ) ) ;
#81520=CARTESIAN_POINT ( 'NONE',  ( -89.25187456871118741, -295.3378472127571968, -216.6496211389093673 ) ) ;
#81521=CARTESIAN_POINT ( 'NONE',  ( -107.4182413264988867, -278.7947956418959734, -238.3222776578252251 ) ) ;
#81522=CARTESIAN_POINT ( 'NONE',  ( -99.66634836054889490, -299.0265852024221545, -229.5621137030160810 ) ) ;
#81525=CARTESIAN_POINT ( 'NONE',  ( -110.8323744494958163, -271.0393599817121526, -250.8442989716325258 ) ) ;
#81527=CARTESIAN_POINT ( 'NONE',  ( -39.16557828376275552, -276.5833071689592089, -343.3998878949193454 ) ) ;
#81528=CARTESIAN_POINT ( 'NONE',  ( -24.24268197716851603, -275.4207735462100572, -194.8325718524619674 ) ) ;
#81529=CARTESIAN_POINT ( 'NONE',  ( 24.90943393627685154, -281.2085776663339516, -315.3013132314085283 ) ) ;
#81530=CARTESIAN_POINT ( 'NONE',  ( -37.24449393671535091, -290.8110606060461123, -344.3743908985322832 ) ) ;
#81531=CARTESIAN_POINT ( 'NONE',  ( -23.53560918908046773, -299.7421508013676430, -194.0509510646687659 ) ) ;
#81532=CARTESIAN_POINT ( 'NONE',  ( -66.75769995234024634, -296.6341364125992186, -341.1050666453737108 ) ) ;
#81533=CARTESIAN_POINT ( 'NONE',  ( -66.05334213155849454, -293.6757415116455263, -201.2410391655178614 ) ) ;
#81534=CARTESIAN_POINT ( 'NONE',  ( 35.09178510338133350, -279.7946907542589656, -289.2115230566017203 ) ) ;
#81535=CARTESIAN_POINT ( 'NONE',  ( -11.26110028518248463, -282.3146674815915276, -200.5849068157895374 ) ) ;
#81536=CARTESIAN_POINT ( 'NONE',  ( -72.32043912949114883, -295.6654774467655784, -204.6366580609269192 ) ) ;
#81537=CARTESIAN_POINT ( 'NONE',  ( -93.34575983112711128, -286.8638263222467799, -218.6118593460829800 ) ) ;
#81538=CARTESIAN_POINT ( 'NONE',  ( 10.30578182832529244, -287.2971193838337740, -326.1412745977937675 ) ) ;
#81539=CARTESIAN_POINT ( 'NONE',  ( -38.25200987741680336, -140.4184747178956343, -364.5570500621696510 ) ) ;
#81541=CARTESIAN_POINT ( 'NONE',  ( -70.40069959264657484, -288.0540586919979660, -339.2645996929285275 ) ) ;
#81542=CARTESIAN_POINT ( 'NONE',  ( 35.57403419954985679, -287.1559421773070540, -265.5895491088462563 ) ) ;
#81544=CARTESIAN_POINT ( 'NONE',  ( -110.3869172541948700, -285.3363969243524139, -293.7686626534448919 ) ) ;
#81545=CARTESIAN_POINT ( 'NONE',  ( -6.523916385703952159, -274.8016836365604831, -204.1617849641908720 ) ) ;
#81546=CARTESIAN_POINT ( 'NONE',  ( -36.36842439695983842, -290.9844209475647858, -193.6634243876421237 ) ) ;
#81547=CARTESIAN_POINT ( 'NONE',  ( 15.68924443910203692, -282.9762888375470880, -326.0480258216661582 ) ) ;
#81548=CARTESIAN_POINT ( 'NONE',  ( 5.776392461285563051, -282.1451928941652909, -207.4044833621010469 ) ) ;
#81549=CARTESIAN_POINT ( 'NONE',  ( -70.45717404443072951, -283.8100457040980586, -339.8673710692067402 ) ) ;
#81551=CARTESIAN_POINT ( 'NONE',  ( -91.29681870373481445, -279.2572502353401092, -221.1895288330605638 ) ) ;
#81552=CARTESIAN_POINT ( 'NONE',  ( -37.37352853689063181, -274.5523547857346784, -345.3611179825600175 ) ) ;
#81553=CARTESIAN_POINT ( 'NONE',  ( 122.3993579641739728, 149.2681047531912952, -263.6619803441950012 ) ) ;
#81554=EDGE_LOOP ( 'NONE', ( #14547, #2400, #78216, #70299 ) ) ;
#81555=CARTESIAN_POINT ( 'NONE',  ( 4.171787011464936690, -278.4913503194197233, -332.6239384301701421 ) ) ;
#81556=CARTESIAN_POINT ( 'NONE',  ( -56.98314758917310030, -168.9463999539727013, -363.9601112268161387 ) ) ;
#81557=CARTESIAN_POINT ( 'NONE',  ( -60.54039684088365192, -297.0918750966832249, -200.9843253510601357 ) ) ;
#81558=CARTESIAN_POINT ( 'NONE',  ( 35.39649021963634823, -292.7416808081691784, -245.1262667562004935 ) ) ;
#81559=CARTESIAN_POINT ( 'NONE',  ( 185.2856823005118372, 260.3293175957331869, -151.1391428729190523 ) ) ;
#81560=CARTESIAN_POINT ( 'NONE',  ( 52.74161837482967741, -297.7338270766273922, -193.9716452598525223 ) ) ;
#81561=CARTESIAN_POINT ( 'NONE',  ( -106.7922364318259270, -288.6231920933798847, -295.3223563613800025 ) ) ;
#81562=CARTESIAN_POINT ( 'NONE',  ( -69.02332783173842756, -297.3336372524170770, -337.5103162485534085 ) ) ;
#81563=CARTESIAN_POINT ( 'NONE',  ( -79.60648291651470743, -286.7832031638206445, -210.1743301218138527 ) ) ;
#81564=ORIENTED_EDGE ( 'NONE', *, *, #60435, .F. ) ;
#81565=CARTESIAN_POINT ( 'NONE',  ( -84.03256058658378436, -296.6170882930271659, -331.3607465515333956 ) ) ;
#81566=CARTESIAN_POINT ( 'NONE',  ( -110.3800281877222034, -285.0011908244450751, -273.6471505607017889 ) ) ;
#81567=CARTESIAN_POINT ( 'NONE',  ( -35.82243785402641834, -296.8657060230561342, -193.7584906295155918 ) ) ;
#81568=CARTESIAN_POINT ( 'NONE',  ( -16.67988201711195728, -293.1153309467529766, -196.3526854063570397 ) ) ;
#81569=CARTESIAN_POINT ( 'NONE',  ( 33.26543502597483126, -293.6547033828719009, -239.7970971671970517 ) ) ;
#81570=CARTESIAN_POINT ( 'NONE',  ( -104.0468533493264118, -290.3181164821702396, -300.1410053159339668 ) ) ;
#81573=CARTESIAN_POINT ( 'NONE',  ( -57.09095328135572345, -299.6605900812083974, -197.1611648092674898 ) ) ;
#81574=CARTESIAN_POINT ( 'NONE',  ( -46.81659624768673211, -272.7293088958181215, -194.3464150530818415 ) ) ;
#81575=CARTESIAN_POINT ( 'NONE',  ( 34.80093529074917313, -280.4451696346272342, -257.7576024673706456 ) ) ;
#81579=CARTESIAN_POINT ( 'NONE',  ( -80.19711561016082157, -277.1228843770078925, -334.3231448457644888 ) ) ;
#81580=CARTESIAN_POINT ( 'NONE',  ( -89.79662402800906307, -271.6963692214894195, -218.4484858658417465 ) ) ;
#81581=CARTESIAN_POINT ( 'NONE',  ( -69.07239738653603922, -281.4907108190378722, -203.2490599355635368 ) ) ;
#81582=CARTESIAN_POINT ( 'NONE',  ( 30.26966211654734451, -274.0980063522423507, -301.0135105961224440 ) ) ;
#81583=CARTESIAN_POINT ( 'NONE',  ( -65.74044477742103254, -298.8772838463473818, -202.6806790964819811 ) ) ;
#81584=CARTESIAN_POINT ( 'NONE',  ( -65.91596933917897161, -274.6101130862098785, -202.9302675682357346 ) ) ;
#81585=CARTESIAN_POINT ( 'NONE',  ( -37.27495885999479697, -299.6530978762457949, -194.1603388541626600 ) ) ;
#81586=CARTESIAN_POINT ( 'NONE',  ( 24.00290855613504704, -272.9796924011017154, -226.5755129491877540 ) ) ;
#81587=CARTESIAN_POINT ( 'NONE',  ( 32.44658160340369335, -294.4915137755492651, -292.1209066123664115 ) ) ;
#81588=CARTESIAN_POINT ( 'NONE',  ( 25.35935763370303420, -291.5989863552330235, -231.7422419614223372 ) ) ;
#81590=CARTESIAN_POINT ( 'NONE',  ( -72.80673558396618716, -278.0014665834356151, -338.6528785617550739 ) ) ;
#81591=CARTESIAN_POINT ( 'NONE',  ( -40.77706564845924930, -274.1745594221836768, -197.3922959930540628 ) ) ;
#81593=CARTESIAN_POINT ( 'NONE',  ( -97.66598511725841547, -282.6042219454085966, -317.4172431457615176 ) ) ;
#81594=CARTESIAN_POINT ( 'NONE',  ( -55.59971727143970810, -297.2867801675276382, -343.2766391937759067 ) ) ;
#81596=CARTESIAN_POINT ( 'NONE',  ( -37.27047264571911001, -285.2501954749469064, -197.1872097385394227 ) ) ;
#81597=CARTESIAN_POINT ( 'NONE',  ( -22.12267351696975481, -280.8574611657795685, -343.9709655066067171 ) ) ;
#81599=CARTESIAN_POINT ( 'NONE',  ( -39.20543821871805790, -275.3157182006963239, -344.3509855061574285 ) ) ;
#81600=CARTESIAN_POINT ( 'NONE',  ( 20.47421352498274061, -274.7641869881182402, -315.9082663212735156 ) ) ;
#81601=CARTESIAN_POINT ( 'NONE',  ( -15.69785892337878508, -282.3322176857517434, -198.4986803509737570 ) ) ;
#81602=CARTESIAN_POINT ( 'NONE',  ( 34.21747475951372053, -276.5424138334703912, -253.9827549142806902 ) ) ;
#81605=CARTESIAN_POINT ( 'NONE',  ( -52.36771837151059117, -272.2628353220592885, -195.6034358290793591 ) ) ;
#81606=CARTESIAN_POINT ( 'NONE',  ( -104.5481009790185851, -280.9972328273689754, -236.5801782912776332 ) ) ;
#81608=CARTESIAN_POINT ( 'NONE',  ( -31.02899395412981320, -288.0514537690238512, -195.0522291287576024 ) ) ;
#81610=CARTESIAN_POINT ( 'NONE',  ( -94.42509389845753276, -289.2256952187570960, -221.6950631401307135 ) ) ;
#81611=CARTESIAN_POINT ( 'NONE',  ( 82.12839394370399759, -301.1616880754598924, -196.5497600369658073 ) ) ;
#81612=CARTESIAN_POINT ( 'NONE',  ( -97.51767341889299701, -294.7643033988899219, -312.3847154461004152 ) ) ;
#81613=CARTESIAN_POINT ( 'NONE',  ( -47.13434429495616484, -290.0660109057705540, -196.7746409711008084 ) ) ;
#81614=CARTESIAN_POINT ( 'NONE',  ( 168.8235619055982113, 230.3815547064285738, -190.2228674158758395 ) ) ;
#81616=CARTESIAN_POINT ( 'NONE',  ( 39.00843874868931493, -286.0471595427563329, -271.5598921398479320 ) ) ;
#81617=CARTESIAN_POINT ( 'NONE',  ( -92.70874832080957617, -282.0720905285465392, -322.4231050419248277 ) ) ;
#81618=CARTESIAN_POINT ( 'NONE',  ( -46.99446503852924906, -291.9261271243483407, -198.0021231748401931 ) ) ;
#81619=CARTESIAN_POINT ( 'NONE',  ( 36.15531568292917797, -283.0256259870450890, -274.0439949215377737 ) ) ;
#81620=CARTESIAN_POINT ( 'NONE',  ( 33.48240068952684823, -282.5972305728804486, -288.7563043430086509 ) ) ;
#81621=CARTESIAN_POINT ( 'NONE',  ( -5.015299507994749995, -290.6086075241711342, -338.4444515369659712 ) ) ;
#81623=CARTESIAN_POINT ( 'NONE',  ( -109.1484134547367404, -273.2385679935342750, -242.4737820105218589 ) ) ;
#81624=CARTESIAN_POINT ( 'NONE',  ( -4.972541508331775439, -286.7091926481447217, -338.6508816839652809 ) ) ;
#81625=CARTESIAN_POINT ( 'NONE',  ( 24.47987131220617840, -274.9418145528446757, -224.4580319789651242 ) ) ;
#81627=CARTESIAN_POINT ( 'NONE',  ( -91.01617433687907521, -293.2650626749801859, -218.4872553857778144 ) ) ;
#81629=CARTESIAN_POINT ( 'NONE',  ( 35.77081079830085031, -289.8376638359844719, -253.6410175316879361 ) ) ;
#81630=CARTESIAN_POINT ( 'NONE',  ( -110.3001379511744773, -276.7843817808888502, -252.2226227578659916 ) ) ;
#81632=CARTESIAN_POINT ( 'NONE',  ( -107.0330269614949827, -295.3508064804711353, -239.4158173966790173 ) ) ;
#81633=CARTESIAN_POINT ( 'NONE',  ( -64.38351344228058792, -293.2934088378746083, -201.6802611414068451 ) ) ;
#81634=CARTESIAN_POINT ( 'NONE',  ( -69.52837777310138279, -272.9654644204912870, -204.7264438328053018 ) ) ;
#81635=CARTESIAN_POINT ( 'NONE',  ( -110.3900185015198758, -292.2043677344128128, -260.2530174932358591 ) ) ;
#81636=CARTESIAN_POINT ( 'NONE',  ( -64.16892672441777279, -292.6346387786325636, -202.2027799395722241 ) ) ;
#81637=CARTESIAN_POINT ( 'NONE',  ( -103.1494808854555032, -286.7664346686281647, -236.4891531330040664 ) ) ;
#81638=CARTESIAN_POINT ( 'NONE',  ( 19.92496197988670303, -294.2868802007924387, -219.7534551073445073 ) ) ;
#81639=CARTESIAN_POINT ( 'NONE',  ( -70.69793139008710625, -292.9365514218004023, -201.5086662383682210 ) ) ;
#81640=CARTESIAN_POINT ( 'NONE',  ( -41.04134257427484300, -294.9332907131907859, -343.2798760160671350 ) ) ;
#81641=CARTESIAN_POINT ( 'NONE',  ( 18.35936030458486812, -288.8521129955078663, -220.1185269631860706 ) ) ;
#81642=CARTESIAN_POINT ( 'NONE',  ( 39.27833376018075029, -281.8208250199415943, -278.5164184276005130 ) ) ;
#81643=CARTESIAN_POINT ( 'NONE',  ( -111.8491326714697180, -270.8700077986529209, -256.3356461168180545 ) ) ;
#81644=CARTESIAN_POINT ( 'NONE',  ( -105.4311018208756394, -284.8510027319231881, -234.2909678048208661 ) ) ;
#81645=CARTESIAN_POINT ( 'NONE',  ( 35.09946729279015187, -277.2997023367249199, -252.3576719530347816 ) ) ;
#81646=CARTESIAN_POINT ( 'NONE',  ( -73.73927684388478099, -284.3523612073391860, -206.6100015843028643 ) ) ;
#81647=CARTESIAN_POINT ( 'NONE',  ( 37.58122927918864065, -285.4955006632043819, -265.9617785773266405 ) ) ;
#81648=CARTESIAN_POINT ( 'NONE',  ( -36.73820996776817083, -278.1992510171389199, -194.5858810721728958 ) ) ;
#81650=CARTESIAN_POINT ( 'NONE',  ( -56.34093780218476866, -282.8113158081263236, -340.9090974665748490 ) ) ;
#81651=CARTESIAN_POINT ( 'NONE',  ( -96.52052592055589741, -280.4141484921134975, -221.7004517271347197 ) ) ;
#81652=CARTESIAN_POINT ( 'NONE',  ( 23.68170821781545499, -285.9878601338201065, -223.7674258250456489 ) ) ;
#81653=CARTESIAN_POINT ( 'NONE',  ( 16.91705418887001144, -296.0258548913882350, -320.6995882996473028 ) ) ;
#81654=CARTESIAN_POINT ( 'NONE',  ( -69.94008744300448654, -279.0744079446678825, -339.2505487498410162 ) ) ;
#81655=CARTESIAN_POINT ( 'NONE',  ( 5.608361393400615569, -277.7986745285733718, -333.6745485249807075 ) ) ;
#81656=CARTESIAN_POINT ( 'NONE',  ( -89.08731883574807853, -277.6379124203764945, -321.9245602074665840 ) ) ;
#81657=CARTESIAN_POINT ( 'NONE',  ( -105.9001735268633553, -274.9215396830576879, -240.7074501944988469 ) ) ;
#81658=CARTESIAN_POINT ( 'NONE',  ( 12.37051056494015100, -284.7456518831746735, -214.3564716067566849 ) ) ;
#81659=CARTESIAN_POINT ( 'NONE',  ( -43.10128925807787681, -290.7238529822260489, -346.3431392017514554 ) ) ;
#81660=CARTESIAN_POINT ( 'NONE',  ( -15.51384472010242810, -293.6833690411612565, -340.3985863505198495 ) ) ;
#81662=CARTESIAN_POINT ( 'NONE',  ( -6.759917655077732235, -294.3059758813359963, -336.6698057062560565 ) ) ;
#81664=CARTESIAN_POINT ( 'NONE',  ( -97.04075038563554756, -290.9836356689590389, -318.5224085003367236 ) ) ;
#81665=CARTESIAN_POINT ( 'NONE',  ( -70.99596869006805377, -280.2472151768046160, -205.4526122486982445 ) ) ;
#81667=CARTESIAN_POINT ( 'NONE',  ( -48.90973313567330649, -296.8285647415410722, -194.4942580596371045 ) ) ;
#81668=CARTESIAN_POINT ( 'NONE',  ( 35.85327613079493858, -288.5004276563072949, -293.9367035957822623 ) ) ;
#81669=CARTESIAN_POINT ( 'NONE',  ( -69.34464197355562476, -289.7951007624710655, -340.3866506129477330 ) ) ;
#81670=CARTESIAN_POINT ( 'NONE',  ( -92.57233954507852047, -284.2048386811063665, -318.1469109438336318 ) ) ;
#81672=CARTESIAN_POINT ( 'NONE',  ( 172.2203992884101069, 243.0707097176554043, -178.6047228861598910 ) ) ;
#81673=CARTESIAN_POINT ( 'NONE',  ( -56.07279955880657951, -169.1889862642364051, -360.6176426954027079 ) ) ;
#81674=CARTESIAN_POINT ( 'NONE',  ( -59.25307663538929859, -276.5403294896335638, -340.1643650859928698 ) ) ;
#81675=CARTESIAN_POINT ( 'NONE',  ( -54.03763492351997400, -276.1917721815169671, -341.7960554523485825 ) ) ;
#81676=CARTESIAN_POINT ( 'NONE',  ( 7.950400138221583646, -298.1126310072594947, -193.4263109806098839 ) ) ;
#81677=CARTESIAN_POINT ( 'NONE',  ( -106.8441832117048875, -265.9836032479844334, -305.8845056521548713 ) ) ;
#81678=CARTESIAN_POINT ( 'NONE',  ( -42.78788612005686076, -275.8043580061844864, -346.6738779317395256 ) ) ;
#81679=CARTESIAN_POINT ( 'NONE',  ( -48.06382480049870054, -289.6844529238566679, -342.6826778869114491 ) ) ;
#81680=CARTESIAN_POINT ( 'NONE',  ( -68.12218479301739649, -298.4611051804134263, -199.9004540013002895 ) ) ;
#81681=CARTESIAN_POINT ( 'NONE',  ( 34.17715015035893344, -286.4586989024804211, -287.2814470124419586 ) ) ;
#81682=CARTESIAN_POINT ( 'NONE',  ( 76.26758135708726627, -299.9312107013272453, -193.4133755750621617 ) ) ;
#81683=CARTESIAN_POINT ( 'NONE',  ( -96.10158266802766036, -297.3261569210868629, -227.0240094179578421 ) ) ;
#81686=CARTESIAN_POINT ( 'NONE',  ( -64.55322078613674819, -279.3246348767544873, -340.9063943174588189 ) ) ;
#81688=CARTESIAN_POINT ( 'NONE',  ( -58.47586977684338194, -282.8257856576762492, -344.3954471951713003 ) ) ;
#81689=CARTESIAN_POINT ( 'NONE',  ( -93.83548717843014231, -278.9720845331555097, -317.0999220533333869 ) ) ;
#81690=CARTESIAN_POINT ( 'NONE',  ( -111.4189468759351342, -280.5268095417676477, -253.4337575196671821 ) ) ;
#81692=CARTESIAN_POINT ( 'NONE',  ( -39.16487771124121764, -296.6035876180735045, -196.7819657958442292 ) ) ;
#81694=CARTESIAN_POINT ( 'NONE',  ( -38.35598725574979539, -280.2057721526154523, -197.3557639725252670 ) ) ;
#81695=CARTESIAN_POINT ( 'NONE',  ( 38.57783508923524352, -276.5076616489199637, -282.5436712995240782 ) ) ;
#81696=CARTESIAN_POINT ( 'NONE',  ( 24.43439190859696808, -278.1297590524230827, -312.9800392277856531 ) ) ;
#81697=CARTESIAN_POINT ( 'NONE',  ( 38.73252060783467243, -274.0298001884705172, -262.6579311392850968 ) ) ;
#81700=CARTESIAN_POINT ( 'NONE',  ( -107.1526404102343548, -290.0392534629336296, -248.4320811874937078 ) ) ;
#81701=CARTESIAN_POINT ( 'NONE',  ( 5.130297916989874807, -285.9584118267812300, -206.1927601651087798 ) ) ;
#81702=CARTESIAN_POINT ( 'NONE',  ( 10.54752895163773196, -280.6203346498940618, -326.8607211160672250 ) ) ;
#81703=CARTESIAN_POINT ( 'NONE',  ( -33.48333667966325322, -281.5773931398748005, -343.8618043847972103 ) ) ;
#81704=CARTESIAN_POINT ( 'NONE',  ( -37.25512277678583928, -284.1330549220610351, -195.9084808381126379 ) ) ;
#81705=CARTESIAN_POINT ( 'NONE',  ( -108.8659954780599008, -292.2592040743076609, -293.0957207673508833 ) ) ;
#81706=CARTESIAN_POINT ( 'NONE',  ( 13.59970718387610766, -281.9898080790516701, -217.4499471845261667 ) ) ;
#81707=CARTESIAN_POINT ( 'NONE',  ( -112.1833100136661585, -270.6240362747285531, -264.7498312333518129 ) ) ;
#81708=CARTESIAN_POINT ( 'NONE',  ( -30.30922140166665812, -281.3644661619290446, -346.2359139161668509 ) ) ;
#81709=CARTESIAN_POINT ( 'NONE',  ( 30.43389058723382945, -295.9762457352487104, -302.5987744817679754 ) ) ;
#81710=CARTESIAN_POINT ( 'NONE',  ( -112.3032331533630952, -276.6343661818296482, -282.8006750906004640 ) ) ;
#81711=CARTESIAN_POINT ( 'NONE',  ( -63.92327072832434709, -287.7064970886273159, -200.0376239088250259 ) ) ;
#81713=CARTESIAN_POINT ( 'NONE',  ( -105.9631163195439854, -292.8860414310746592, -238.6070255444787165 ) ) ;
#81714=CARTESIAN_POINT ( 'NONE',  ( 35.52370789363173031, -273.7807801508527064, -288.1812025981160446 ) ) ;
#81716=CARTESIAN_POINT ( 'NONE',  ( -62.71998869198446158, -288.5712730437087430, -342.9439427101294768 ) ) ;
#81717=CARTESIAN_POINT ( 'NONE',  ( -17.19484027032354945, -290.7162995976032676, -199.3111526025095657 ) ) ;
#81719=CARTESIAN_POINT ( 'NONE',  ( -51.39145209629101174, -275.9204033576540951, -342.4988192647832079 ) ) ;
#81720=CARTESIAN_POINT ( 'NONE',  ( -111.4438894342690674, -294.7493514445453684, -265.9191569274854032 ) ) ;
#81721=CARTESIAN_POINT ( 'NONE',  ( -88.99585677463919353, -291.1122554514721514, -322.6400963451912958 ) ) ;
#81724=CARTESIAN_POINT ( 'NONE',  ( 30.27890819409663337, -292.4923626002055244, -305.7187349992332770 ) ) ;
#81725=CARTESIAN_POINT ( 'NONE',  ( 2.865992995962707734, -288.2018570862796309, -208.4758868868453305 ) ) ;
#81726=CARTESIAN_POINT ( 'NONE',  ( 31.93176170945120163, -286.1962301827105080, -301.5886938793698278 ) ) ;
#81727=CARTESIAN_POINT ( 'NONE',  ( 15.43957754999853194, -288.2419125267824711, -219.0823539217273606 ) ) ;
#81730=CARTESIAN_POINT ( 'NONE',  ( 28.95197012942375991, -287.9380140802033452, -239.4135654103442050 ) ) ;
#81731=CARTESIAN_POINT ( 'NONE',  ( -22.39852171518658963, -296.8416151114992090, -344.2198224035504381 ) ) ;
#81733=CARTESIAN_POINT ( 'NONE',  ( 24.37421298961141858, -288.1513152695231952, -224.9832071944996699 ) ) ;
#81734=CARTESIAN_POINT ( 'NONE',  ( -26.01050746721648466, -274.9887816967616914, -345.0666617444682061 ) ) ;
#81735=CARTESIAN_POINT ( 'NONE',  ( -25.76895742779925058, -277.2418540313242374, -346.4650989418158247 ) ) ;
#81736=CARTESIAN_POINT ( 'NONE',  ( -94.94314872069300293, -278.9109482867825136, -219.2943243530987445 ) ) ;
#81737=CARTESIAN_POINT ( 'NONE',  ( -106.2909426827863513, -298.9070820918510663, -241.7630629577626564 ) ) ;
#81738=CARTESIAN_POINT ( 'NONE',  ( -97.35129869781235357, -283.1666775117235488, -225.3739116760270633 ) ) ;
#81740=CARTESIAN_POINT ( 'NONE',  ( -77.46996165711199467, -277.6475204092960212, -207.8451630430427315 ) ) ;
#81741=CARTESIAN_POINT ( 'NONE',  ( -19.42160838525141742, -280.8216104449914496, -343.2423238295277201 ) ) ;
#81743=CARTESIAN_POINT ( 'NONE',  ( -23.08757232357777411, -275.3530328817878399, -345.3783213572709201 ) ) ;
#81744=CARTESIAN_POINT ( 'NONE',  ( -109.1570256572031781, -298.2882931683211041, -253.8303353658724006 ) ) ;
#81746=CARTESIAN_POINT ( 'NONE',  ( -47.23017728899625922, -282.0953262108982358, -346.4118282267479572 ) ) ;
#81747=CARTESIAN_POINT ( 'NONE',  ( -109.5097604275956797, -297.6572095929784609, -257.9040107300236286 ) ) ;
#81748=CARTESIAN_POINT ( 'NONE',  ( -68.61960193026243360, -275.0743771140536751, -200.6309853788793589 ) ) ;
#81749=CARTESIAN_POINT ( 'NONE',  ( -92.92712001049940795, -272.8924114127940470, -222.9883748504422840 ) ) ;
#81750=CARTESIAN_POINT ( 'NONE',  ( 7.861940942577713365, -294.6698512480499517, -210.5143847409766806 ) ) ;
#81751=CARTESIAN_POINT ( 'NONE',  ( 37.37631310072897861, -287.4860428834808772, -251.7541702567963000 ) ) ;
#81752=CARTESIAN_POINT ( 'NONE',  ( -106.0984352063183991, -277.0416037779816634, -238.9011393139275583 ) ) ;
#81753=CARTESIAN_POINT ( 'NONE',  ( -114.2514034051426108, -290.3388494518025595, -274.0890592805192227 ) ) ;
#81754=CARTESIAN_POINT ( 'NONE',  ( -48.10737545686681926, -288.2510845727973106, -342.8519951788838966 ) ) ;
#81755=CARTESIAN_POINT ( 'NONE',  ( 23.21506827447304744, -290.9489093193146232, -226.1131976733700526 ) ) ;
#81757=CARTESIAN_POINT ( 'NONE',  ( 193.6056169066500274, 279.7126221763799094, -126.0203154767880989 ) ) ;
#81758=CARTESIAN_POINT ( 'NONE',  ( -98.34746959362136920, -290.6180054286815562, -230.0661910540931103 ) ) ;
#81761=CARTESIAN_POINT ( 'NONE',  ( -110.7047327889479362, -285.7801002085042228, -247.5837576834900062 ) ) ;
#81762=CARTESIAN_POINT ( 'NONE',  ( -0.9049426016482470247, -291.5826589218674485, -202.7949806477763559 ) ) ;
#81763=CARTESIAN_POINT ( 'NONE',  ( 37.94331977287701818, -283.0396546585653823, -284.0524904631643039 ) ) ;
#81764=CARTESIAN_POINT ( 'NONE',  ( 1.099503359059319951, -282.3570541274576158, -332.4787756473494369 ) ) ;
#81765=CARTESIAN_POINT ( 'NONE',  ( -113.3895472435426512, -296.7041695495339582, -258.2059314512890751 ) ) ;
#81766=CARTESIAN_POINT ( 'NONE',  ( 28.29425190653734035, -276.4215915415323366, -237.2980679554437415 ) ) ;
#81767=CARTESIAN_POINT ( 'NONE',  ( -22.38699921989589114, -290.2646919169902731, -197.2297039364170530 ) ) ;
#81768=CARTESIAN_POINT ( 'NONE',  ( -31.29176557035528461, -272.9251503415742377, -197.2010906507908032 ) ) ;
#81771=CARTESIAN_POINT ( 'NONE',  ( -33.18217398097159077, -288.0249575611264845, -195.9866133404147206 ) ) ;
#81772=CARTESIAN_POINT ( 'NONE',  ( -95.33868696863227399, -296.9512037699159350, -320.5392210541604072 ) ) ;
#81773=CARTESIAN_POINT ( 'NONE',  ( -87.77080910989245410, -285.9760027947467051, -217.4385553528673825 ) ) ;
#81774=CARTESIAN_POINT ( 'NONE',  ( -65.02145387072246763, -276.4636904490992038, -342.0178748278774492 ) ) ;
#81775=CARTESIAN_POINT ( 'NONE',  ( 24.72726607723750547, -293.6000544971045088, -224.9655651053417955 ) ) ;
#81776=CARTESIAN_POINT ( 'NONE',  ( 35.19584521420294720, -285.9713246467692329, -292.2832870148955067 ) ) ;
#81777=CARTESIAN_POINT ( 'NONE',  ( -22.09758208446846695, -295.1952691141890455, -345.8154827105825007 ) ) ;
#81778=CARTESIAN_POINT ( 'NONE',  ( -72.64089133273367338, -291.9046863170812003, -206.3820421999429300 ) ) ;
#81781=CARTESIAN_POINT ( 'NONE',  ( 193.8404912567452811, 275.6304219182297288, -124.1201750204255347 ) ) ;
#81782=CARTESIAN_POINT ( 'NONE',  ( -110.4381947116660569, -285.7944235713907233, -292.3064571030392358 ) ) ;
#81783=CARTESIAN_POINT ( 'NONE',  ( 44.71564893372296723, -279.0523547857346784, -270.3937649182068412 ) ) ;
#81786=CARTESIAN_POINT ( 'NONE',  ( -107.6924227151188518, -283.2003506976758445, -291.0215416415543359 ) ) ;
#81787=CARTESIAN_POINT ( 'NONE',  ( -113.7457979206378127, -278.0961323147606095, -280.1725934299769278 ) ) ;
#81788=CARTESIAN_POINT ( 'NONE',  ( 16.56273339335434969, -282.8204410233846602, -218.3800833316968237 ) ) ;
#81789=CARTESIAN_POINT ( 'NONE',  ( 105.0249005777022830, 114.6126997019200360, -281.5807060078374207 ) ) ;
#81791=CARTESIAN_POINT ( 'NONE',  ( -33.10966586809888668, -281.5745935888664917, -346.6676397022843048 ) ) ;
#81792=CARTESIAN_POINT ( 'NONE',  ( 30.31108749893536825, -285.1557371353844132, -238.8183355138148158 ) ) ;
#81793=CARTESIAN_POINT ( 'NONE',  ( -80.56546497701046405, -275.3338081803476030, -208.0720400864513806 ) ) ;
#81794=CARTESIAN_POINT ( 'NONE',  ( -105.0165476886413529, -296.6759819436445014, -297.8947964356850662 ) ) ;
#81795=CARTESIAN_POINT ( 'NONE',  ( -36.18165813180068113, -290.7517847617235702, -196.8645606999143354 ) ) ;
#81796=CARTESIAN_POINT ( 'NONE',  ( -114.2760003891828546, -279.2238068309048344, -268.7446783730263746 ) ) ;
#81797=CARTESIAN_POINT ( 'NONE',  ( -3.867466406026852432, -276.5976231072189648, -335.2338832752563462 ) ) ;
#81798=CARTESIAN_POINT ( 'NONE',  ( -106.5701162009084726, -274.0565483484143670, -237.3623465369909411 ) ) ;
#81799=CARTESIAN_POINT ( 'NONE',  ( 39.32222630230873506, -274.4469488364879339, -268.3276743101127977 ) ) ;
#81800=CARTESIAN_POINT ( 'NONE',  ( -114.0438498157189002, -273.6021558389782058, -270.3744870444270418 ) ) ;
#81801=CARTESIAN_POINT ( 'NONE',  ( -1.969472082924502709, -274.5836062597261389, -336.5102494578166556 ) ) ;
#81802=CARTESIAN_POINT ( 'NONE',  ( 0.2664318177568268387, -295.9867744330525738, -336.8911040734342350 ) ) ;
#81805=CARTESIAN_POINT ( 'NONE',  ( -110.4027120996655498, -285.5526695175209966, -276.3872778473191829 ) ) ;
#81806=CARTESIAN_POINT ( 'NONE',  ( -106.0793285600362594, -285.8918550963797998, -302.7511233675093081 ) ) ;
#81807=CARTESIAN_POINT ( 'NONE',  ( 20.42629911730043801, -286.2706687486016790, -225.5643443071005265 ) ) ;
#81808=CARTESIAN_POINT ( 'NONE',  ( -29.65008982035340068, -275.3531513455819777, -343.8106704035644725 ) ) ;
#81809=CARTESIAN_POINT ( 'NONE',  ( 34.15537272895061705, -283.6721949639400009, -290.3369547551836831 ) ) ;
#81810=CARTESIAN_POINT ( 'NONE',  ( -105.9200193510129537, -276.6746724043322274, -297.3374387780215784 ) ) ;
#81811=CARTESIAN_POINT ( 'NONE',  ( 18.55297594529989524, -277.3034173617404008, -317.7954015868837701 ) ) ;
#81813=CARTESIAN_POINT ( 'NONE',  ( -56.88410069332447705, -274.2857279978143197, -199.9089025418762446 ) ) ;
#81814=CARTESIAN_POINT ( 'NONE',  ( -3.737478874769393666, -281.2871097864644412, -201.2458706343960841 ) ) ;
#81815=CARTESIAN_POINT ( 'NONE',  ( -31.08502114258416427, -280.6214083127929371, -193.6248278700684295 ) ) ;
#81819=CARTESIAN_POINT ( 'NONE',  ( -1.573939786598276491, -288.3815594679065839, -203.5706036674124562 ) ) ;
#81820=CARTESIAN_POINT ( 'NONE',  ( -110.4034589047474810, -295.6990532250833894, -274.1796426937573301 ) ) ;
#81821=CARTESIAN_POINT ( 'NONE',  ( -94.62982060207428958, -290.5975093576415134, -219.0641001426003811 ) ) ;
#81822=CARTESIAN_POINT ( 'NONE',  ( 36.14165336782868820, -286.1130108396071137, -276.5587328561424556 ) ) ;
#81823=CARTESIAN_POINT ( 'NONE',  ( -69.02800365246380920, -288.0520120069662084, -336.7791357795305771 ) ) ;
#81824=CARTESIAN_POINT ( 'NONE',  ( -67.72600776497776565, -286.8493510531387756, -203.5485117216191782 ) ) ;
#81825=CARTESIAN_POINT ( 'NONE',  ( -66.94330246224842540, -275.4399410940307007, -339.2722621481120200 ) ) ;
#81826=CARTESIAN_POINT ( 'NONE',  ( -29.08433485324762202, -287.3491754652595773, -346.1653662221929721 ) ) ;
#81827=CARTESIAN_POINT ( 'NONE',  ( 10.77445444981035827, -288.7170840278666901, -212.7621915810391044 ) ) ;
#81828=CARTESIAN_POINT ( 'NONE',  ( 9.075335884246451101, -286.4169884501742445, -329.5499619058292069 ) ) ;
#81830=CARTESIAN_POINT ( 'NONE',  ( 5.740147648839000638, -283.3931850303210354, -329.5841104735433760 ) ) ;
#81831=CARTESIAN_POINT ( 'NONE',  ( -112.4188885866651333, -292.5053411525380511, -274.0277509019301760 ) ) ;
#81832=CARTESIAN_POINT ( 'NONE',  ( 82.16616378849288083, -298.1952514025611549, -193.8821863655754782 ) ) ;
#81834=CARTESIAN_POINT ( 'NONE',  ( -107.5596446376046345, -298.8346440975439577, -242.3142239576204702 ) ) ;
#81835=CARTESIAN_POINT ( 'NONE',  ( -27.52661224193222012, -279.3770542723340213, -197.8097042457567625 ) ) ;
#81836=CARTESIAN_POINT ( 'NONE',  ( 36.54158805151680411, -279.3864321950910607, -257.4669185781934289 ) ) ;
#81837=CARTESIAN_POINT ( 'NONE',  ( 15.36048956961786693, -293.5269951826068677, -326.2774664076555382 ) ) ;
#81838=CARTESIAN_POINT ( 'NONE',  ( -50.07210710525713893, -296.2868542674112291, -197.6673964413452893 ) ) ;
#81839=CARTESIAN_POINT ( 'NONE',  ( 31.60265774430837027, -274.0023605277337992, -298.5693183149202810 ) ) ;
#81840=CARTESIAN_POINT ( 'NONE',  ( -45.12643243768917500, -296.4678364360436831, -343.4916276328756339 ) ) ;
#81842=CARTESIAN_POINT ( 'NONE',  ( -94.63257186325374448, -271.8168149200270705, -219.8006362846780064 ) ) ;
#81843=CARTESIAN_POINT ( 'NONE',  ( -112.1376571302561871, -294.9618256313630695, -256.9619078844593218 ) ) ;
#81844=CARTESIAN_POINT ( 'NONE',  ( 13.29556812846294989, -294.2026951447872989, -216.9640957840976796 ) ) ;
#81846=CARTESIAN_POINT ( 'NONE',  ( -1.185750365669597128, -293.3478312319411430, -206.7435534227670928 ) ) ;
#81848=CARTESIAN_POINT ( 'NONE',  ( -109.5395023486533148, -282.2949744204166223, -291.9903268073858840 ) ) ;
#81849=CARTESIAN_POINT ( 'NONE',  ( -35.65061426688678381, -295.0303824265330945, -343.3540239828761287 ) ) ;
#81850=CARTESIAN_POINT ( 'NONE',  ( -52.91761354190613531, -283.2463447877308909, -345.8237721711282120 ) ) ;
#81851=CARTESIAN_POINT ( 'NONE',  ( 35.92879161800063059, -283.2369343717919605, -251.9017236092358587 ) ) ;
#81852=CARTESIAN_POINT ( 'NONE',  ( -89.86871470747274770, -285.0017514214624157, -214.0155652234949173 ) ) ;
#81853=CARTESIAN_POINT ( 'NONE',  ( -93.02061219355790911, -289.2502622922914952, -220.3430877252356765 ) ) ;
#81854=CARTESIAN_POINT ( 'NONE',  ( 21.06670925402145045, -280.6992485220796993, -319.4647376872765108 ) ) ;
#81855=CARTESIAN_POINT ( 'NONE',  ( -27.75575714261201199, -284.8612592378886461, -197.4958095402900256 ) ) ;
#81857=CARTESIAN_POINT ( 'NONE',  ( 39.04809207600354881, -286.3800592629153812, -263.0006598632234613 ) ) ;
#81859=CARTESIAN_POINT ( 'NONE',  ( 21.16980649560883876, -295.7785865678103505, -315.3578538571466083 ) ) ;
#81860=CARTESIAN_POINT ( 'NONE',  ( -110.8685469066999048, -279.7147891454112028, -291.1555666755861580 ) ) ;
#81861=CARTESIAN_POINT ( 'NONE',  ( 25.13367469356369099, -292.1395384917993852, -312.4946479065531548 ) ) ;
#81862=CARTESIAN_POINT ( 'NONE',  ( -72.13604744183439266, -279.2451302517991962, -206.1626687658101389 ) ) ;
#81863=CARTESIAN_POINT ( 'NONE',  ( 23.10675043577578691, -293.0806612251284946, -222.6432482840647822 ) ) ;
#81864=CARTESIAN_POINT ( 'NONE',  ( -46.30986967815339028, -284.0190521048506866, -195.3352149116694250 ) ) ;
#81865=CARTESIAN_POINT ( 'NONE',  ( -83.61196066571294239, -279.6866015623040198, -329.4530489213889837 ) ) ;
#81866=CARTESIAN_POINT ( 'NONE',  ( -92.37538662734166905, -294.9233904793816805, -318.6798700241328106 ) ) ;
#81867=CARTESIAN_POINT ( 'NONE',  ( -40.33426559960402358, -296.0145062507014586, -195.3700666537613131 ) ) ;
#81870=CARTESIAN_POINT ( 'NONE',  ( 25.04363643110249171, -282.9751916411251500, -229.2811638800966989 ) ) ;
#81871=CARTESIAN_POINT ( 'NONE',  ( -110.1109977801522604, -296.1530367031302262, -263.2874672295286587 ) ) ;
#81873=CARTESIAN_POINT ( 'NONE',  ( -20.19161114001082069, -277.7666405000204009, -195.3683826091709363 ) ) ;
#81874=CARTESIAN_POINT ( 'NONE',  ( -58.06820870452099115, -272.9882866742243550, -196.3154697137528615 ) ) ;
#81875=CARTESIAN_POINT ( 'NONE',  ( 28.48799599358683921, -289.3784775099378521, -309.3450811002564933 ) ) ;
#81876=CARTESIAN_POINT ( 'NONE',  ( -66.33098238309098349, -289.2757625204578744, -337.4123104797594692 ) ) ;
#81877=CARTESIAN_POINT ( 'NONE',  ( -100.0679635560566538, -280.6017478704646919, -231.5839706051217206 ) ) ;
#81878=CARTESIAN_POINT ( 'NONE',  ( -108.7190306916724722, -274.3995554054992567, -251.4108339425437748 ) ) ;
#81879=CARTESIAN_POINT ( 'NONE',  ( -101.1494763215244888, -277.8411810278536791, -234.0885636033075912 ) ) ;
#81881=CARTESIAN_POINT ( 'NONE',  ( 1.197259963528528148, -274.3852407785665832, -203.6843853388399452 ) ) ;
#81882=CARTESIAN_POINT ( 'NONE',  ( -22.47650772332466929, -294.1641104950489307, -197.4204554565887690 ) ) ;
#81884=CARTESIAN_POINT ( 'NONE',  ( -108.8119729918828256, -291.4058927102275902, -255.0023170748712573 ) ) ;
#81886=CARTESIAN_POINT ( 'NONE',  ( 12.48426344257400444, -290.8774155372340147, -213.2850386474827360 ) ) ;
#81887=CONICAL_SURFACE ( 'NONE', #38088, 5.751884811727114410, 0.09862129276975223346 ) ;
#81888=CARTESIAN_POINT ( 'NONE',  ( -93.62715280958242658, -296.8783414987095171, -223.8224746449104714 ) ) ;
#81891=CARTESIAN_POINT ( 'NONE',  ( -95.14845873381477759, -292.7511371824128332, -220.5306347086738867 ) ) ;
#81892=CARTESIAN_POINT ( 'NONE',  ( -37.37352853689063181, -288.5519495502701375, -190.3611179825600175 ) ) ;
#81894=CARTESIAN_POINT ( 'NONE',  ( 5.761052669849259011, -288.6375055859787722, -209.1243513350736123 ) ) ;
#81895=CARTESIAN_POINT ( 'NONE',  ( -26.78750629475706191, -274.9174345947448614, -344.4464567279875382 ) ) ;
#81896=CARTESIAN_POINT ( 'NONE',  ( 22.62701544133324205, -276.8663004806123809, -226.2582002445645912 ) ) ;
#81897=CARTESIAN_POINT ( 'NONE',  ( -34.78378499846022720, -290.1643845635553589, -195.9650746031211952 ) ) ;
#81898=CARTESIAN_POINT ( 'NONE',  ( -81.53784422453607306, -281.3181985650274441, -208.8224608222790266 ) ) ;
#81900=CARTESIAN_POINT ( 'NONE',  ( 25.64264714001457079, -281.4108975866635660, -307.5672530217617577 ) ) ;
#81901=CARTESIAN_POINT ( 'NONE',  ( -112.6950455080724254, -279.8117695599299282, -256.0301802651289336 ) ) ;
#81902=CARTESIAN_POINT ( 'NONE',  ( 29.40832813381082289, -280.8384585780484599, -308.0516618248084342 ) ) ;
#81903=CARTESIAN_POINT ( 'NONE',  ( -11.93272297255542114, -277.6707218386073919, -342.8544650504663309 ) ) ;
#81905=CARTESIAN_POINT ( 'NONE',  ( -34.15172917704009592, -275.6117045972064830, -194.1211557628172670 ) ) ;
#81906=CARTESIAN_POINT ( 'NONE',  ( -37.30987171927208124, -279.5519495502701375, -340.3611179825599606 ) ) ;
#81909=CARTESIAN_POINT ( 'NONE',  ( -102.9768132442638802, -299.0350594075123922, -234.0701745892964709 ) ) ;
#81910=CARTESIAN_POINT ( 'NONE',  ( -109.2392014585838638, -291.4429157286500640, -284.7422280120297842 ) ) ;
#81911=CARTESIAN_POINT ( 'NONE',  ( 7.356775695287544714, -290.2126114348805004, -331.8753478756458435 ) ) ;
#81912=CARTESIAN_POINT ( 'NONE',  ( -41.59047878508010854, -291.3459532735535049, -197.3328449412940984 ) ) ;
#81913=CARTESIAN_POINT ( 'NONE',  ( 16.63830924949025913, -287.8171335449700337, -325.2593285999844284 ) ) ;
#81915=CARTESIAN_POINT ( 'NONE',  ( -93.17760984515453515, -282.2717416064941744, -318.6379106467322231 ) ) ;
#81916=CARTESIAN_POINT ( 'NONE',  ( -108.9103891702190907, -292.1541548040448220, -290.2680375753525936 ) ) ;
#81917=CARTESIAN_POINT ( 'NONE',  ( -109.3381587566622386, -283.2382603741286289, -254.5791156361851222 ) ) ;
#81918=CARTESIAN_POINT ( 'NONE',  ( 36.01104725288168851, -282.8078356335022363, -265.8204210585134888 ) ) ;
#81919=CARTESIAN_POINT ( 'NONE',  ( 16.52940227328300082, -289.2505017365108415, -325.1225646238522131 ) ) ;
#81920=CARTESIAN_POINT ( 'NONE',  ( -110.4129375776936826, -279.0767773678546746, -267.9124500087638125 ) ) ;
#81921=CARTESIAN_POINT ( 'NONE',  ( -76.95074138161147914, -290.3293231260586822, -204.7321783276440215 ) ) ;
#81922=CARTESIAN_POINT ( 'NONE',  ( -40.81941977351774398, -286.8124147291862300, -193.5492517992728665 ) ) ;
#81923=CARTESIAN_POINT ( 'NONE',  ( 7.502970291046463736, -287.1378008828476709, -207.7776469902497070 ) ) ;
#81924=CARTESIAN_POINT ( 'NONE',  ( -108.9293832670439741, -284.9073413963066628, -256.0711345212769174 ) ) ;
#81927=CARTESIAN_POINT ( 'NONE',  ( 31.06044012695905110, -294.9867342045036480, -237.6593316390317625 ) ) ;
#81928=CARTESIAN_POINT ( 'NONE',  ( 38.36640547815856905, -292.0937119227294261, -258.9787496378156675 ) ) ;
#81929=CARTESIAN_POINT ( 'NONE',  ( 5.524836989298125722, -275.5146758498975714, -329.8027580354513475 ) ) ;
#81930=CARTESIAN_POINT ( 'NONE',  ( -35.46665834869380518, -297.4236408775723817, -193.4632510446849096 ) ) ;
#81931=CARTESIAN_POINT ( 'NONE',  ( 25.00358950345557929, -292.5708276532235459, -309.7478065793825408 ) ) ;
#81932=CARTESIAN_POINT ( 'NONE',  ( -84.70635495581396412, -295.6292443764529594, -213.4209975048893000 ) ) ;
#81933=CARTESIAN_POINT ( 'NONE',  ( -108.1389300001882816, -292.0116532427509810, -250.9992289203728433 ) ) ;
#81934=CARTESIAN_POINT ( 'NONE',  ( 21.23253139735124151, -294.0153737215701995, -226.2784062279527859 ) ) ;
#81936=CARTESIAN_POINT ( 'NONE',  ( 20.85073852395589711, -292.2064657978497166, -317.9593404461119235 ) ) ;
#81937=CARTESIAN_POINT ( 'NONE',  ( -84.48606600356380625, -299.4036879818700072, -211.9649669003583483 ) ) ;
#81938=CARTESIAN_POINT ( 'NONE',  ( 35.89057345946819311, -288.5021574104857791, -271.0263642303369807 ) ) ;
#81939=CARTESIAN_POINT ( 'NONE',  ( 33.65988051194787545, -277.8593400264110755, -295.7575412167898321 ) ) ;
#81940=CARTESIAN_POINT ( 'NONE',  ( -93.05580144302479084, -276.6248595587082377, -323.0105112299098664 ) ) ;
#81941=CARTESIAN_POINT ( 'NONE',  ( -68.79477288089572085, -272.9980274141841505, -200.1754024032130985 ) ) ;
#81942=CARTESIAN_POINT ( 'NONE',  ( 19.57998248787507123, -280.3005101761426090, -318.3520991093543557 ) ) ;
#81943=CARTESIAN_POINT ( 'NONE',  ( -105.6375096225134911, -276.5117870389955783, -304.2752045577215654 ) ) ;
#81944=CARTESIAN_POINT ( 'NONE',  ( -110.8778073330106224, -295.2226525680596296, -271.4538477544599004 ) ) ;
#81945=CARTESIAN_POINT ( 'NONE',  ( -111.5779681219408417, -274.6939240792844430, -259.3321695784418921 ) ) ;
#81946=CARTESIAN_POINT ( 'NONE',  ( -76.62598443508069579, -274.1624624771984600, -208.7118059462517579 ) ) ;
#81949=CARTESIAN_POINT ( 'NONE',  ( -100.2956681714494778, -289.1296890515407085, -228.8524962540716672 ) ) ;
#81950=CARTESIAN_POINT ( 'NONE',  ( -48.87334312926287794, -273.7346232423334413, -198.2265123423171929 ) ) ;
#81952=CARTESIAN_POINT ( 'NONE',  ( 39.57763484180127023, -287.4953391697130769, -265.8183967183750269 ) ) ;
#81953=CARTESIAN_POINT ( 'NONE',  ( -106.4033990180104325, -274.9410280707010088, -240.5559909656385855 ) ) ;
#81954=CARTESIAN_POINT ( 'NONE',  ( -73.02055219059077729, -293.5259162891216533, -336.1560482086745765 ) ) ;
#81955=CARTESIAN_POINT ( 'NONE',  ( -52.89494398800645314, -282.4436414019826884, -345.6634568889118668 ) ) ;
#81958=CARTESIAN_POINT ( 'NONE',  ( 33.92109166633409245, -279.2480669793171728, -246.8177455318251248 ) ) ;
#81960=CARTESIAN_POINT ( 'NONE',  ( -88.19469969223784744, -290.1160943373806163, -217.3654477346387353 ) ) ;
#81961=CARTESIAN_POINT ( 'NONE',  ( -69.56642910586073469, -281.6204821026560694, -337.2514034628729860 ) ) ;
#81964=CARTESIAN_POINT ( 'NONE',  ( -111.1515960138788301, -288.3811207849422544, -283.6690073778734700 ) ) ;
#81965=CARTESIAN_POINT ( 'NONE',  ( -81.50181328099357358, -274.9594527702330424, -211.3005300510968425 ) ) ;
#81966=CARTESIAN_POINT ( 'NONE',  ( -50.01263738428759353, -284.4153233897258133, -345.9624212027071053 ) ) ;
#81967=CARTESIAN_POINT ( 'NONE',  ( -1.953843752632816511, -272.5969758135981920, -203.6002475459519303 ) ) ;
#81968=CARTESIAN_POINT ( 'NONE',  ( -91.66504558039827089, -283.8540456108374315, -319.1444035656863889 ) ) ;
#81969=CARTESIAN_POINT ( 'NONE',  ( 22.95901602566664934, -277.5619691003940375, -312.6291777055037073 ) ) ;
#81970=CARTESIAN_POINT ( 'NONE',  ( 32.25493520775901146, -276.6536211955946101, -292.9201533543655955 ) ) ;
#81971=CARTESIAN_POINT ( 'NONE',  ( -52.48814562653897298, -285.2461834197364396, -343.8688423207035498 ) ) ;
#81974=CARTESIAN_POINT ( 'NONE',  ( 23.17035501552031107, -294.0224567087636842, -317.9983529183751898 ) ) ;
#81975=CARTESIAN_POINT ( 'NONE',  ( 36.62250982825553791, -289.3974439777578027, -259.9275491606242667 ) ) ;
#81977=CARTESIAN_POINT ( 'NONE',  ( -72.02372285203398405, -295.1237833571632336, -198.2697987213421698 ) ) ;
#81978=CARTESIAN_POINT ( 'NONE',  ( -99.98851142236988210, -278.0602045213016140, -226.1245997568183839 ) ) ;
#81979=CARTESIAN_POINT ( 'NONE',  ( 1.312049252156952672, -290.9588973335400510, -204.6324907156576955 ) ) ;
#81980=CARTESIAN_POINT ( 'NONE',  ( -46.83317061714643614, -287.4497245803039505, -197.2303155561596668 ) ) ;
#81982=CARTESIAN_POINT ( 'NONE',  ( -91.69701426713092474, -279.5999645334164825, -320.6698298519895616 ) ) ;
#81983=CARTESIAN_POINT ( 'NONE',  ( -43.63596989400259929, -287.3995043910445020, -194.1571762311504870 ) ) ;
#81984=CARTESIAN_POINT ( 'NONE',  ( 28.62596424251758620, -284.0261726310041013, -306.0439976796699852 ) ) ;
#81985=CARTESIAN_POINT ( 'NONE',  ( -6.572750981931142711, -276.8258589327974732, -340.9605836434483308 ) ) ;
#81986=CARTESIAN_POINT ( 'NONE',  ( -106.0532071854996161, -270.9421275412298087, -240.5860623452868481 ) ) ;
#81987=CARTESIAN_POINT ( 'NONE',  ( -113.2361289795359198, -278.5480729526414621, -257.3597459846866400 ) ) ;
#81989=CARTESIAN_POINT ( 'NONE',  ( -68.67552125017202513, -299.5572776468279130, -202.8230691811378961 ) ) ;
#81992=CARTESIAN_POINT ( 'NONE',  ( -4.771743288812468897, -279.1233781216988064, -337.9199732462171255 ) ) ;
#81993=CARTESIAN_POINT ( 'NONE',  ( -90.74778589981694665, -295.4440507633330526, -216.6201142531493247 ) ) ;
#81995=CARTESIAN_POINT ( 'NONE',  ( -92.77741965935388180, -277.3828267383703974, -317.9517624608558322 ) ) ;
#81996=CARTESIAN_POINT ( 'NONE',  ( -67.39407707522751423, -274.8717218198938212, -199.8993314660514216 ) ) ;
#81997=CARTESIAN_POINT ( 'NONE',  ( 27.65852530215709493, -280.0734236964347588, -229.4228801387190799 ) ) ;
#81998=CARTESIAN_POINT ( 'NONE',  ( -5.334197129653129643, -290.3852100296180652, -337.0956200676806702 ) ) ;
#81999=CARTESIAN_POINT ( 'NONE',  ( -102.5132835257025903, -297.5492595903598954, -310.0520800404493684 ) ) ;
#82000=CARTESIAN_POINT ( 'NONE',  ( -113.8363059277430551, -297.6947739397306805, -275.3289945141840462 ) ) ;
#82001=CARTESIAN_POINT ( 'NONE',  ( 31.53337820212854226, -295.1675051219065722, -240.9668696124453220 ) ) ;
#82002=CARTESIAN_POINT ( 'NONE',  ( 37.39565679682894483, -279.6007446362789324, -274.1500365170583677 ) ) ;
#82003=CARTESIAN_POINT ( 'NONE',  ( -41.14881242091294666, -281.9240118109325977, -196.0185319670774504 ) ) ;
#82004=CARTESIAN_POINT ( 'NONE',  ( -39.17984955077309195, -296.1087858823657371, -195.9311581210084228 ) ) ;
#82005=CARTESIAN_POINT ( 'NONE',  ( -113.5276546315382831, -286.1926276178770649, -267.1684642221741228 ) ) ;
#82006=CARTESIAN_POINT ( 'NONE',  ( 33.69148388100780522, -286.2336494736513828, -252.1854886667417190 ) ) ;
#82007=CARTESIAN_POINT ( 'NONE',  ( -98.09277876945984076, -248.9093811562096903, -333.9997278395424019 ) ) ;
#82009=CARTESIAN_POINT ( 'NONE',  ( 29.83594339479149582, -286.6028097845501179, -306.8828598634932519 ) ) ;
#82010=CARTESIAN_POINT ( 'NONE',  ( 17.79494098031452154, -286.5365691460364701, -222.4858812299608815 ) ) ;
#82012=CARTESIAN_POINT ( 'NONE',  ( -111.9153293960401072, -285.4064035991736432, -288.3126544640929296 ) ) ;
#82013=CARTESIAN_POINT ( 'NONE',  ( 11.55753433926364870, -275.0860068397330451, -216.0624895750014787 ) ) ;
#82015=CARTESIAN_POINT ( 'NONE',  ( -66.88361849078992805, -290.5942973018921975, -199.5884709384627627 ) ) ;
#82016=CARTESIAN_POINT ( 'NONE',  ( 38.04725899704824599, -282.3934068725969837, -285.5208550841853707 ) ) ;
#82017=CARTESIAN_POINT ( 'NONE',  ( -88.48125708762592012, -280.8704605134516896, -213.7267338582360310 ) ) ;
#82018=CARTESIAN_POINT ( 'NONE',  ( 39.59880616501320816, -281.9158260488990777, -272.7906823057586507 ) ) ;
#82019=CARTESIAN_POINT ( 'NONE',  ( 7.142324975062856574, -280.6772154670964028, -212.4164943776545442 ) ) ;
#82020=CARTESIAN_POINT ( 'NONE',  ( 30.89617123739170168, -291.2666405000203440, -285.9686137636504668 ) ) ;
#82021=CARTESIAN_POINT ( 'NONE',  ( -113.3215480562446658, -274.3158145202488072, -270.3835736289650526 ) ) ;
#82023=CARTESIAN_POINT ( 'NONE',  ( 6.490750052572844098, -278.4556149095211026, -331.0777790653958732 ) ) ;
#82024=CARTESIAN_POINT ( 'NONE',  ( -71.96233075983749927, -195.6174374264305413, -359.8130507035538130 ) ) ;
#82025=CARTESIAN_POINT ( 'NONE',  ( 37.16309042514302519, -279.5132999550452837, -265.7913275264203321 ) ) ;
#82026=CARTESIAN_POINT ( 'NONE',  ( -90.11371190002310527, -296.6304481117311980, -219.7020522695422073 ) ) ;
#82027=CARTESIAN_POINT ( 'NONE',  ( 1.674307107433533837, -292.0664998206391374, -203.9882551612451209 ) ) ;
#82030=CARTESIAN_POINT ( 'NONE',  ( -40.39836935881152158, -296.5893015249340010, -193.9597787784593663 ) ) ;
#82031=CARTESIAN_POINT ( 'NONE',  ( -110.4179503107032616, -288.8162978539924666, -280.7622457466610513 ) ) ;
#82032=CARTESIAN_POINT ( 'NONE',  ( -108.7852277242770498, -298.1504164546531115, -290.5276210609516738 ) ) ;
#82033=CARTESIAN_POINT ( 'NONE',  ( -8.073843208075505373, -287.7589408186571518, -202.9472022800918865 ) ) ;
#82035=CARTESIAN_POINT ( 'NONE',  ( 15.26815831641564003, -293.7144415564771407, -214.3862379636885862 ) ) ;
#82037=CARTESIAN_POINT ( 'NONE',  ( -109.6740326450353393, -285.1802179702024205, -260.0644139302452231 ) ) ;
#82038=CARTESIAN_POINT ( 'NONE',  ( -89.32751306955358928, -296.1348258943406222, -214.0266428071479652 ) ) ;
#82039=CARTESIAN_POINT ( 'NONE',  ( -39.21801796046428024, -292.8320275124491445, -193.5324982138299390 ) ) ;
#82040=CARTESIAN_POINT ( 'NONE',  ( -94.66964200860503809, -291.7410850516274081, -219.0480204045339008 ) ) ;
#82041=CARTESIAN_POINT ( 'NONE',  ( -90.59130243329686039, -289.9995744522460654, -320.3696907042939301 ) ) ;
#82044=CARTESIAN_POINT ( 'NONE',  ( -94.65256039330974147, -299.0935287128514801, -220.7270525447967202 ) ) ;
#82045=CARTESIAN_POINT ( 'NONE',  ( -96.61899181487805777, -272.0021148594323108, -221.8204370528361835 ) ) ;
#82046=CARTESIAN_POINT ( 'NONE',  ( 34.56755605576303481, -280.4276044773031913, -256.4217376337435326 ) ) ;
#82048=CARTESIAN_POINT ( 'NONE',  ( -2.758393568358715964, -276.1149841649949508, -339.1036660766311002 ) ) ;
#82049=CARTESIAN_POINT ( 'NONE',  ( -111.1417001269576730, -270.9522812833232024, -270.3407916626836709 ) ) ;
#82050=CARTESIAN_POINT ( 'NONE',  ( -99.03308318034230240, -280.9775889039833601, -228.9776851961528621 ) ) ;
#82051=CARTESIAN_POINT ( 'NONE',  ( -71.03423050132707317, -275.6412904287990386, -336.5100324117742048 ) ) ;
#82052=CARTESIAN_POINT ( 'NONE',  ( -79.97106840304445541, -298.6658550758359638, -210.6127501027602875 ) ) ;
#82053=CARTESIAN_POINT ( 'NONE',  ( 95.09830598555298309, -300.8281214179230574, -197.0271103297674813 ) ) ;
#82054=CARTESIAN_POINT ( 'NONE',  ( -80.19216316353535490, -299.0830228283499537, -207.2875222114244025 ) ) ;
#82055=CARTESIAN_POINT ( 'NONE',  ( 0.3940681800939942470, -272.5723212446074513, -205.1202525051882333 ) ) ;
#82056=CARTESIAN_POINT ( 'NONE',  ( 21.07025797407371570, -293.5871847924900067, -226.4073261193454698 ) ) ;
#82057=CARTESIAN_POINT ( 'NONE',  ( 23.08204006807817521, -291.5458836830696328, -228.3347825882860036 ) ) ;
#82059=CARTESIAN_POINT ( 'NONE',  ( -31.44871836864349746, -277.4721050401014395, -347.1261470677173406 ) ) ;
#82060=CARTESIAN_POINT ( 'NONE',  ( -56.86365599382574487, -273.9601132543831454, -199.9671383623970371 ) ) ;
#82061=CARTESIAN_POINT ( 'NONE',  ( -3.128495950987585150, -281.2945866025168016, -338.8063339251074240 ) ) ;
#82063=CARTESIAN_POINT ( 'NONE',  ( -27.95100427542504917, -296.9334926527635048, -344.9909090803030267 ) ) ;
#82065=CARTESIAN_POINT ( 'NONE',  ( -61.59788182152129821, -282.5725472605432174, -339.4379448474290939 ) ) ;
#82066=CARTESIAN_POINT ( 'NONE',  ( -95.76396267262362016, -281.9020240531446575, -317.6768880052978830 ) ) ;
#82067=CARTESIAN_POINT ( 'NONE',  ( 16.01269113468555361, -274.8516610959954960, -321.0433027240094361 ) ) ;
#82068=CARTESIAN_POINT ( 'NONE',  ( -2.946393120940041577, -282.5067821597840521, -203.6988334198388486 ) ) ;
#82071=CARTESIAN_POINT ( 'NONE',  ( -49.57055690205050524, -272.2987273795579881, -195.0955372750555341 ) ) ;
#82072=CARTESIAN_POINT ( 'NONE',  ( -110.9281324447398873, -280.7495242648145108, -254.9671001587985302 ) ) ;
#82074=CARTESIAN_POINT ( 'NONE',  ( -1.671352019772091246, -288.4412879387947442, -203.7507549311218895 ) ) ;
#82076=CARTESIAN_POINT ( 'NONE',  ( -104.7567830899720605, -288.1174226417805926, -303.3445663842726958 ) ) ;
#82078=CARTESIAN_POINT ( 'NONE',  ( -109.2769426472226684, -295.1550138320130259, -284.9994838495284739 ) ) ;
#82079=CARTESIAN_POINT ( 'NONE',  ( 20.46059208423668707, -286.3393909041870415, -316.9418060296706585 ) ) ;
#82080=CARTESIAN_POINT ( 'NONE',  ( 196.7445862410842778, 294.2657832282549748, -82.73034305482168804 ) ) ;
#82081=CARTESIAN_POINT ( 'NONE',  ( -78.59127603965620779, -295.4969896299979268, -207.6610904924703220 ) ) ;
#82082=CARTESIAN_POINT ( 'NONE',  ( 36.70872738699967641, -285.7995137569665189, -251.9425963325003863 ) ) ;
#82083=CARTESIAN_POINT ( 'NONE',  ( 28.87780597464708876, -283.5903332957850580, -303.0565577872225163 ) ) ;
#82084=CARTESIAN_POINT ( 'NONE',  ( -30.33099509431403717, -281.2044791313864494, -346.0236848713168456 ) ) ;
#82085=CARTESIAN_POINT ( 'NONE',  ( -108.7105680981734679, -290.7545849382271967, -255.0156077379456292 ) ) ;
#82087=CARTESIAN_POINT ( 'NONE',  ( 23.07884904121814529, -283.5582309932527210, -312.3698332182628405 ) ) ;
#82088=CARTESIAN_POINT ( 'NONE',  ( 32.38833408974344508, -282.6498862780698005, -292.6694504346328927 ) ) ;
#82089=CARTESIAN_POINT ( 'NONE',  ( 22.00795887290809105, -290.1663917648011193, -316.8149171160421247 ) ) ;
#82090=AXIS2_PLACEMENT_3D ( 'NONE', #20503, #42247, #5369 ) ;
#82091=CARTESIAN_POINT ( 'NONE',  ( 7.986968146524043632, -298.7716743175183751, -193.3598638625616957 ) ) ;
#82093=CARTESIAN_POINT ( 'NONE',  ( 38.73575424438563886, -275.7049586598034239, -282.5794011309642997 ) ) ;
#82094=CARTESIAN_POINT ( 'NONE',  ( -0.4655609963800500517, -294.5247008367717285, -205.4464179428558737 ) ) ;
#82096=CARTESIAN_POINT ( 'NONE',  ( -20.25526795762937127, -282.7662352645560304, -195.3538533559490702 ) ) ;
#82098=CARTESIAN_POINT ( 'NONE',  ( 33.46518172348125830, -273.8799286651936313, -295.7416329638515435 ) ) ;
#82100=CARTESIAN_POINT ( 'NONE',  ( -109.0906698790647624, -295.2793660700268106, -244.6993613384723005 ) ) ;
#82101=CARTESIAN_POINT ( 'NONE',  ( -68.15356948044015439, -293.2407799932713601, -203.2870407263492893 ) ) ;
#82102=CARTESIAN_POINT ( 'NONE',  ( 0.6725464450685151307, -273.9222637228679105, -207.9206685476900986 ) ) ;
#82104=CARTESIAN_POINT ( 'NONE',  ( -69.33596237181502886, -293.1435359469183481, -203.9613785948843656 ) ) ;
#82105=CARTESIAN_POINT ( 'NONE',  ( -44.33456818686888568, -292.9029330361613006, -197.4094620365269463 ) ) ;
#82106=CARTESIAN_POINT ( 'NONE',  ( -111.2414875306717761, -286.3765952599508182, -265.4195759632858085 ) ) ;
#82107=CARTESIAN_POINT ( 'NONE',  ( -112.0675905779172155, -292.1792724512033033, -254.3416348630592267 ) ) ;
#82108=CARTESIAN_POINT ( 'NONE',  ( -6.103715620221827898, -293.7692909668433003, -200.5079179685447741 ) ) ;
#82109=CARTESIAN_POINT ( 'NONE',  ( 20.52190693189797344, -294.0120640264001963, -314.8877966234297219 ) ) ;
#82110=CARTESIAN_POINT ( 'NONE',  ( 34.58086250074265422, -289.2779139203096861, -249.0521506466539563 ) ) ;
#82111=CARTESIAN_POINT ( 'NONE',  ( 6.926743768686855596, -282.6348991959138743, -333.4287393679612705 ) ) ;
#82112=CARTESIAN_POINT ( 'NONE',  ( -32.01114943876781638, -296.1982380766883693, -194.8028378855136964 ) ) ;
#82113=CARTESIAN_POINT ( 'NONE',  ( -111.4920438856211007, -284.1254119646054050, -291.1150700196210437 ) ) ;
#82114=AXIS2_PLACEMENT_3D ( 'NONE', #82546, #47006, #22564 ) ;
#82115=CARTESIAN_POINT ( 'NONE',  ( 35.50384725203758762, -277.7429538309397685, -286.7096000896301575 ) ) ;
#82116=ADVANCED_FACE ( 'NONE', ( #88971 ), #12604, .T. ) ;
#82117=CARTESIAN_POINT ( 'NONE',  ( -99.37480345308760832, -282.8067672581210559, -309.6866999271533132 ) ) ;
#82118=CARTESIAN_POINT ( 'NONE',  ( 36.33050929770327997, -285.3715910787586267, -256.3109859636529109 ) ) ;
#82119=CARTESIAN_POINT ( 'NONE',  ( -111.8552238822559701, -276.5165395997362339, -284.1452945737259483 ) ) ;
#82121=CARTESIAN_POINT ( 'NONE',  ( -26.74003697949952496, -282.4214522944017745, -342.7007248049748682 ) ) ;
#82123=CARTESIAN_POINT ( 'NONE',  ( -28.28724677181754643, -281.3695499766986927, -194.2418413332855209 ) ) ;
#82124=CARTESIAN_POINT ( 'NONE',  ( 36.15663519833373840, -286.8903402198855588, -292.5610913724917168 ) ) ;
#82125=CARTESIAN_POINT ( 'NONE',  ( -28.75648742360392873, -296.7021008025943161, -343.9265685650195223 ) ) ;
#82126=CARTESIAN_POINT ( 'NONE',  ( 19.42611638585554346, -276.4548932462366793, -219.4519631878720531 ) ) ;
#82127=CARTESIAN_POINT ( 'NONE',  ( -10.53619142669411879, -275.7096897475483388, -198.6475026056864124 ) ) ;
#82128=CARTESIAN_POINT ( 'NONE',  ( -96.09426739027080089, -277.7779894194200665, -313.7079971486831482 ) ) ;
#82129=CARTESIAN_POINT ( 'NONE',  ( -110.7518782995152691, -274.7100404944453658, -256.5640544879563549 ) ) ;
#82130=CARTESIAN_POINT ( 'NONE',  ( 30.48204292126207449, -285.1354721065071658, -238.7388425717042537 ) ) ;
#82131=CARTESIAN_POINT ( 'NONE',  ( -104.4417740241912327, -291.6804689559690473, -306.4723419537276072 ) ) ;
#82133=CARTESIAN_POINT ( 'NONE',  ( 20.75981818490537378, -293.0992203979575379, -315.0855773402889781 ) ) ;
#82135=CARTESIAN_POINT ( 'NONE',  ( -70.22643930907140941, -291.2730325280579677, -205.1638679189195216 ) ) ;
#82137=CARTESIAN_POINT ( 'NONE',  ( -62.64862278765789938, -290.4534736357731504, -342.8123836119005432 ) ) ;
#82138=CARTESIAN_POINT ( 'NONE',  ( -109.7239409426571086, -279.3429944211504221, -259.7771122502529693 ) ) ;
#82140=CARTESIAN_POINT ( 'NONE',  ( -80.43990177356813831, -296.4036545708666495, -206.8619732081066900 ) ) ;
#82141=CARTESIAN_POINT ( 'NONE',  ( 34.75577602402540123, -287.8649821034501315, -243.6166471730477099 ) ) ;
#82142=CARTESIAN_POINT ( 'NONE',  ( 38.95374992914764789, -287.7573982976631441, -260.1264420195140588 ) ) ;
#82143=CARTESIAN_POINT ( 'NONE',  ( -107.4110120342696604, -284.6130751241904022, -290.9576144652219796 ) ) ;
#82144=CARTESIAN_POINT ( 'NONE',  ( -112.7898643569067900, -271.0197764341745597, -296.3298465391405330 ) ) ;
#82145=CARTESIAN_POINT ( 'NONE',  ( 192.2886581304107096, 278.8240533624382351, -125.2388310753975418 ) ) ;
#82146=CARTESIAN_POINT ( 'NONE',  ( 44.79179776835351845, 11.33544171671844580, -328.3433051430387195 ) ) ;
#82148=CARTESIAN_POINT ( 'NONE',  ( -80.92374628910054923, -276.8584106975106920, -329.1251118808432352 ) ) ;
#82149=CARTESIAN_POINT ( 'NONE',  ( -108.2681701242387220, -277.7167875131541450, -251.7737250035820864 ) ) ;
#82150=CARTESIAN_POINT ( 'NONE',  ( -26.21448397584709156, -297.6956243422372950, -193.4235562049308612 ) ) ;
#82151=CARTESIAN_POINT ( 'NONE',  ( 202.7398265782193221, 290.0209625311386503, -82.55066922910880578 ) ) ;
#82152=CARTESIAN_POINT ( 'NONE',  ( -8.088789376390691288, -275.3617651508644713, -341.0687710340085346 ) ) ;
#82154=CARTESIAN_POINT ( 'NONE',  ( -108.9978554447150003, -290.8556865092985504, -284.6863532519028013 ) ) ;
#82155=CARTESIAN_POINT ( 'NONE',  ( -37.26403528140092902, -298.8559311974310617, -193.5218205314156137 ) ) ;
#82156=CARTESIAN_POINT ( 'NONE',  ( 34.19417533085546523, -286.0154989581392329, -253.4584735647162290 ) ) ;
#82157=CARTESIAN_POINT ( 'NONE',  ( -83.52550538733954966, -274.0891177587608354, -208.8097631244746140 ) ) ;
#82158=CARTESIAN_POINT ( 'NONE',  ( -47.79093832560312194, -295.3552761443186228, -342.6606740253980661 ) ) ;
#82160=CARTESIAN_POINT ( 'NONE',  ( -106.2525905069612833, -280.0674473281030714, -301.4819427822596367 ) ) ;
#82161=CARTESIAN_POINT ( 'NONE',  ( 25.05370473753441374, -281.6574099407159224, -315.3983698282480077 ) ) ;
#82164=CARTESIAN_POINT ( 'NONE',  ( -110.7012053438168380, -279.6279966159377750, -270.6529480603770139 ) ) ;
#82165=CARTESIAN_POINT ( 'NONE',  ( -112.0047537040155845, -280.4921293873322838, -256.1704305727635642 ) ) ;
#82166=CARTESIAN_POINT ( 'NONE',  ( -82.28978495796707193, -296.0000757693032369, -212.0295361154890941 ) ) ;
#82168=CARTESIAN_POINT ( 'NONE',  ( -94.79217245488219135, -279.3540500217516751, -225.3027557184658463 ) ) ;
#82170=CARTESIAN_POINT ( 'NONE',  ( -2.639636848006202907, -275.3020532080696512, -201.7904432705693694 ) ) ;
#82171=CARTESIAN_POINT ( 'NONE',  ( 37.62171321351074482, -286.4294392609133979, -285.6511452717745101 ) ) ;
#82172=CARTESIAN_POINT ( 'NONE',  ( -4.719667921906985697, -276.4819619247717242, -202.8132667201391826 ) ) ;
#82173=CARTESIAN_POINT ( 'NONE',  ( 30.01501722445966536, -274.5980689000616053, -306.5515775254915525 ) ) ;
#82176=CARTESIAN_POINT ( 'NONE',  ( -110.4681864251881507, -289.7026469068417214, -273.9066104233913848 ) ) ;
#82177=CARTESIAN_POINT ( 'NONE',  ( -102.8356115009131031, -283.3733664604519049, -310.6582687441062944 ) ) ;
#82178=CARTESIAN_POINT ( 'NONE',  ( 8.402911710312698901, -280.6563475136866259, -328.6107861503588765 ) ) ;
#82179=CARTESIAN_POINT ( 'NONE',  ( -4.065012856411942543, -279.0745545272598633, -204.7114752265621291 ) ) ;
#82180=CARTESIAN_POINT ( 'NONE',  ( -46.88573168073287434, -284.0100027414964075, -196.4836983738666163 ) ) ;
#82181=CARTESIAN_POINT ( 'NONE',  ( -16.17990006150293780, -290.7788601638627028, -342.3672611418575116 ) ) ;
#82182=CARTESIAN_POINT ( 'NONE',  ( -49.22120863500471444, -281.1024542151716901, -197.9317884155463503 ) ) ;
#82183=CARTESIAN_POINT ( 'NONE',  ( -101.0074826914384971, -271.0844958151715218, -230.7168399829901091 ) ) ;
#82184=CARTESIAN_POINT ( 'NONE',  ( -31.71589676564785165, -281.3821648384673608, -346.3662920569153698 ) ) ;
#82185=CARTESIAN_POINT ( 'NONE',  ( 36.84216627480963524, -295.6939918879463676, -281.3953653382101834 ) ) ;
#82187=CARTESIAN_POINT ( 'NONE',  ( -106.4875885432006726, -277.2015908731663103, -238.7254681870155082 ) ) ;
#82188=CARTESIAN_POINT ( 'NONE',  ( -107.9165083132562586, -278.9522213974703391, -289.4160154648022854 ) ) ;
#82189=CARTESIAN_POINT ( 'NONE',  ( -67.13079451278326815, -285.4419288387170468, -339.3729885893371261 ) ) ;
#82191=CARTESIAN_POINT ( 'NONE',  ( -93.65474649989067757, -293.1686613232927243, -219.9810127070461476 ) ) ;
#82192=CARTESIAN_POINT ( 'NONE',  ( -32.31117604997904635, -274.9886833389989533, -345.2435600996745961 ) ) ;
#82193=CARTESIAN_POINT ( 'NONE',  ( 36.22782511701549879, -287.0287372871783305, -292.5807393657402145 ) ) ;
#82194=CARTESIAN_POINT ( 'NONE',  ( -34.80964736120277792, -290.4843585089363955, -196.6045648799531875 ) ) ;
#82196=CARTESIAN_POINT ( 'NONE',  ( 34.06169929642377525, -274.4656557973740405, -287.8151726627178846 ) ) ;
#82197=CARTESIAN_POINT ( 'NONE',  ( -64.03490053994069342, -293.5434939620507748, -339.6856312753361635 ) ) ;
#82198=CARTESIAN_POINT ( 'NONE',  ( -105.5646293371883360, -291.5023805375322468, -297.8266441504850945 ) ) ;
#82200=CARTESIAN_POINT ( 'NONE',  ( 38.53885564606073189, -291.9242801084453163, -261.8229028761807058 ) ) ;
#82201=CARTESIAN_POINT ( 'NONE',  ( -104.2189597646516432, -286.5705348472563401, -239.0329722847220637 ) ) ;
#82202=CARTESIAN_POINT ( 'NONE',  ( -26.31405430414769242, -287.1534919365759038, -345.5433302373552351 ) ) ;
#82204=CARTESIAN_POINT ( 'NONE',  ( 31.51959912646978879, -288.6321722757145380, -244.2655592401592344 ) ) ;
#82206=CARTESIAN_POINT ( 'NONE',  ( 16.08541515327904392, -287.6373231571927249, -220.3611861522408901 ) ) ;
#82207=CARTESIAN_POINT ( 'NONE',  ( -55.64582352358044659, -297.2665151344614856, -343.4594481038606659 ) ) ;
#82209=CARTESIAN_POINT ( 'NONE',  ( -32.34771155020516886, -287.3188496449234890, -193.9080509642015215 ) ) ;
#82210=CARTESIAN_POINT ( 'NONE',  ( -64.59887507751042790, -275.4849463048752796, -340.8887702656103897 ) ) ;
#82211=CARTESIAN_POINT ( 'NONE',  ( -93.31570017795620231, -278.1629683249696541, -323.2831854781044854 ) ) ;
#82213=CARTESIAN_POINT ( 'NONE',  ( 1.367014395040615948, -280.2208655637672905, -203.7618696849826563 ) ) ;
#82214=CARTESIAN_POINT ( 'NONE',  ( -110.0855082842366102, -298.7479889569253828, -253.6223849895250453 ) ) ;
#82215=CARTESIAN_POINT ( 'NONE',  ( -102.7226632636031525, -283.0426510472877339, -233.5079086041955634 ) ) ;
#82217=CARTESIAN_POINT ( 'NONE',  ( -57.42499831240692743, -277.9297467150012153, -198.8941563019513126 ) ) ;
#82218=CARTESIAN_POINT ( 'NONE',  ( -69.63273108474551520, -281.4769820148094936, -338.0678196151921497 ) ) ;
#82220=CARTESIAN_POINT ( 'NONE',  ( -28.69896665040271344, -275.4244658673873687, -346.2298475127841471 ) ) ;
#82221=CARTESIAN_POINT ( 'NONE',  ( -101.8305640059499666, -298.5550981857519446, -234.6974924434329353 ) ) ;
#82222=CARTESIAN_POINT ( 'NONE',  ( -38.74074939013102181, -281.9896487476350444, -347.0392450602047916 ) ) ;
#82223=CARTESIAN_POINT ( 'NONE',  ( -104.9841060373679795, -297.8686091136740970, -242.2913233571277374 ) ) ;
#82224=CARTESIAN_POINT ( 'NONE',  ( -109.3921034050367922, -298.1941986321468789, -244.6310254897033190 ) ) ;
#82225=CARTESIAN_POINT ( 'NONE',  ( 21.50073740742153916, -274.6132294701671412, -227.1216102180505914 ) ) ;
#82226=CARTESIAN_POINT ( 'NONE',  ( 19.98939996131778685, -294.8835905186925288, -222.0067426427277724 ) ) ;
#82227=CARTESIAN_POINT ( 'NONE',  ( 32.86574627786668401, -288.1227413223216445, -301.9825422648518156 ) ) ;
#82228=CARTESIAN_POINT ( 'NONE',  ( -58.86806092695453430, -277.8556478550650581, -197.9323254586728638 ) ) ;
#82229=CARTESIAN_POINT ( 'NONE',  ( -112.3167853997882304, -290.6048716608109430, -252.8186953152983847 ) ) ;
#82230=CARTESIAN_POINT ( 'NONE',  ( -110.5420538426909189, -289.5642497742517207, -273.9084403105201773 ) ) ;
#82231=CARTESIAN_POINT ( 'NONE',  ( 34.78790591727006642, -291.2869794194224369, -249.7638253195496816 ) ) ;
#82233=CARTESIAN_POINT ( 'NONE',  ( 121.1498776811041438, 150.0802918209077177, -263.8330885344481658 ) ) ;
#82235=CARTESIAN_POINT ( 'NONE',  ( 35.18454678552089376, -287.1761590439653560, -279.1890254501961408 ) ) ;
#82237=CARTESIAN_POINT ( 'NONE',  ( -109.0787770382201103, -285.1447895710801390, -297.8333793970257375 ) ) ;
#82238=CARTESIAN_POINT ( 'NONE',  ( 30.69595308386004007, -292.1495782416866973, -234.6981213144351841 ) ) ;
#82239=CARTESIAN_POINT ( 'NONE',  ( 34.85670431790524049, -282.5442070462915467, -244.8911605663836326 ) ) ;
#82240=CARTESIAN_POINT ( 'NONE',  ( -18.73768537273358348, -282.6392845644988938, -341.0031145581434089 ) ) ;
#82241=CARTESIAN_POINT ( 'NONE',  ( -112.6004999004516378, -296.7565056689679182, -254.0172837666562771 ) ) ;
#82243=CARTESIAN_POINT ( 'NONE',  ( -101.1542196670626623, -274.3647325816482407, -233.8004663928502964 ) ) ;
#82244=CARTESIAN_POINT ( 'NONE',  ( -19.65860351893262248, -290.3006097881522010, -197.7876357410340233 ) ) ;
#82245=CARTESIAN_POINT ( 'NONE',  ( 21.00648153819410879, -273.7240670479724258, -225.8138015972125743 ) ) ;
#82248=CARTESIAN_POINT ( 'NONE',  ( -70.64824542843378197, -287.5296596061101013, -203.7737172930530676 ) ) ;
#82250=CARTESIAN_POINT ( 'NONE',  ( -19.34641712159132965, -295.9056945844068878, -344.9655158664165242 ) ) ;
#82251=CARTESIAN_POINT ( 'NONE',  ( -99.11273405775577316, -284.6629569783329998, -309.5484746508861917 ) ) ;
#82252=CARTESIAN_POINT ( 'NONE',  ( 39.38765851782513749, -274.6571107568639150, -274.0446642464561364 ) ) ;
#82253=CARTESIAN_POINT ( 'NONE',  ( 34.36476604325291362, -293.8495615741924212, -242.4381990131205953 ) ) ;
#82254=CARTESIAN_POINT ( 'NONE',  ( 31.59810485164540239, -285.2820247840532488, -238.8084931115682537 ) ) ;
#82255=CARTESIAN_POINT ( 'NONE',  ( 28.09019071872619122, -294.4170334845036905, -311.0126208583176322 ) ) ;
#82256=CARTESIAN_POINT ( 'NONE',  ( -75.87629644515328664, -289.9156054348987936, -332.3866963630273972 ) ) ;
#82260=CARTESIAN_POINT ( 'NONE',  ( -97.62287679132212759, -246.6820661265134618, -331.3632087810060511 ) ) ;
#82261=CARTESIAN_POINT ( 'NONE',  ( -69.51827648917475244, -287.1564686476422708, -201.1560164551064247 ) ) ;
#82262=CARTESIAN_POINT ( 'NONE',  ( 13.84574458161073807, -272.1952119285918457, -206.2264541496106460 ) ) ;
#82264=CARTESIAN_POINT ( 'NONE',  ( -99.29961629950494739, -282.9321513775680046, -309.6409040358457219 ) ) ;
#82265=CARTESIAN_POINT ( 'NONE',  ( -102.0815077564833047, -277.6711939574131520, -312.1057407934236494 ) ) ;
#82266=CARTESIAN_POINT ( 'NONE',  ( 25.20109864939744426, -282.9954566653009920, -229.1772441344316178 ) ) ;
#82267=CARTESIAN_POINT ( 'NONE',  ( 123.5090149810071409, 147.7087541737730589, -262.2547634134738814 ) ) ;
#82268=CARTESIAN_POINT ( 'NONE',  ( -93.97473387653838017, -282.4245377288726218, -321.6767844689586013 ) ) ;
#82269=CARTESIAN_POINT ( 'NONE',  ( 1.035469685148925123, -284.5867330593611655, -206.2771044218037275 ) ) ;
#82270=CARTESIAN_POINT ( 'NONE',  ( -95.10165138745190916, -275.0844489056009365, -221.3095783874864821 ) ) ;
#82271=CARTESIAN_POINT ( 'NONE',  ( -95.64965695262473844, -296.4263334051639163, -314.4063843879839624 ) ) ;
#82274=CARTESIAN_POINT ( 'NONE',  ( 11.26946036199136891, -291.4269564559353967, -215.1733394214647603 ) ) ;
#82275=CARTESIAN_POINT ( 'NONE',  ( -71.51808368431464658, -278.1431766711897353, -339.2471658741003466 ) ) ;
#82276=CARTESIAN_POINT ( 'NONE',  ( 31.11831592997810603, -275.2142228917865623, -245.0189357298367554 ) ) ;
#82277=CARTESIAN_POINT ( 'NONE',  ( 24.11168832294763575, -275.0853003909469408, -316.2411088120010163 ) ) ;
#82279=CARTESIAN_POINT ( 'NONE',  ( 34.30264110741431693, -273.2639606469523414, -248.0078303435984424 ) ) ;
#82281=CARTESIAN_POINT ( 'NONE',  ( -22.19645008584052803, -296.2870844745876866, -345.2558954538642979 ) ) ;
#82284=CARTESIAN_POINT ( 'NONE',  ( -108.3894215080576373, -285.3943564332374194, -288.4289723431415382 ) ) ;
#82285=CARTESIAN_POINT ( 'NONE',  ( -100.5634172967669571, -285.7489543623862573, -312.6098302468755605 ) ) ;
#82286=CARTESIAN_POINT ( 'NONE',  ( -96.00850166457308887, -283.2898546975542331, -313.9741787090850380 ) ) ;
#82287=CARTESIAN_POINT ( 'NONE',  ( -70.83387214650075236, -275.9015358793878931, -336.1236820343060003 ) ) ;
#82288=CARTESIAN_POINT ( 'NONE',  ( 1.771926599659222168, -284.3838233492475638, -333.5162375429878239 ) ) ;
#82289=CARTESIAN_POINT ( 'NONE',  ( -16.20030696877190479, -275.2538314592206916, -341.0103004042298380 ) ) ;
#82290=CARTESIAN_POINT ( 'NONE',  ( -16.27895970187977426, -277.8532062922993191, -340.6324934970108416 ) ) ;
#82292=CARTESIAN_POINT ( 'NONE',  ( -111.5776778699178209, -279.6043489408739902, -250.4815674253345605 ) ) ;
#82293=CARTESIAN_POINT ( 'NONE',  ( -14.25220602997345587, -280.8359709879707680, -196.9131516146023841 ) ) ;
#82295=ORIENTED_EDGE ( 'NONE', *, *, #33928, .T. ) ;
#82297=CARTESIAN_POINT ( 'NONE',  ( 35.60175027823817118, -289.6739781245664744, -290.8918786898855160 ) ) ;
#82298=CARTESIAN_POINT ( 'NONE',  ( -82.03469701510771017, -296.6224153325352404, -212.3733665212719472 ) ) ;
#82299=CARTESIAN_POINT ( 'NONE',  ( -65.41754804382519239, -288.7581548384026178, -342.0069105027736214 ) ) ;
#82300=CARTESIAN_POINT ( 'NONE',  ( 34.01207602265371577, -285.5357545185896129, -250.6986500786932481 ) ) ;
#82301=CARTESIAN_POINT ( 'NONE',  ( 7.298654567911541768, -285.2485953140867991, -211.7936144675054777 ) ) ;
#82302=CARTESIAN_POINT ( 'NONE',  ( -107.9251798957282631, -288.4988496950435888, -292.8006498307749439 ) ) ;
#82303=CARTESIAN_POINT ( 'NONE',  ( -86.00080711093296770, -286.5653003968828330, -215.3439092773986374 ) ) ;
#82304=CARTESIAN_POINT ( 'NONE',  ( -53.71996759329717719, -275.2620294225641260, -343.6041849123693623 ) ) ;
#82305=CARTESIAN_POINT ( 'NONE',  ( -8.554443554831648200, -287.0815046340810568, -340.9282941819097914 ) ) ;
#82307=CARTESIAN_POINT ( 'NONE',  ( 23.07660013466603388, -288.9462714987811864, -225.9243129156368184 ) ) ;
#82308=CARTESIAN_POINT ( 'NONE',  ( 15.04027593969662391, -284.7889119940051614, -216.4523338357290640 ) ) ;
#82309=CARTESIAN_POINT ( 'NONE',  ( 34.93771068095600185, -282.6484886582146032, -282.1549817048996260 ) ) ;
#82310=CARTESIAN_POINT ( 'NONE',  ( -104.3808280628871898, -293.0019800063693083, -236.2494582837441897 ) ) ;
#82313=CARTESIAN_POINT ( 'NONE',  ( -59.74490947996399370, -299.6844623816042485, -198.1442386401996600 ) ) ;
#82314=CARTESIAN_POINT ( 'NONE',  ( -49.15794227921451665, -279.0948691807164437, -198.1601612854873622 ) ) ;
#82315=CARTESIAN_POINT ( 'NONE',  ( 35.40147729201559201, -279.3168326698464057, -252.0487799954543959 ) ) ;
#82316=CARTESIAN_POINT ( 'NONE',  ( 0.4521515363631591899, -293.7590292533312208, -337.2775621255710803 ) ) ;
#82317=CARTESIAN_POINT ( 'NONE',  ( -106.3530803599599750, -271.1461859268238186, -243.4728301319110813 ) ) ;
#82318=CARTESIAN_POINT ( 'NONE',  ( 33.21268639048580695, -279.9666248977115401, -249.7863270577234402 ) ) ;
#82319=CARTESIAN_POINT ( 'NONE',  ( -57.22314067331819132, -271.8736150133341880, -198.5714445264189862 ) ) ;
#82320=CARTESIAN_POINT ( 'NONE',  ( -28.82229586794989018, -296.2572052988252267, -343.4101705109846421 ) ) ;
#82321=CARTESIAN_POINT ( 'NONE',  ( -35.82564250435292053, -296.5506922128299720, -194.0548301270989100 ) ) ;
#82322=CARTESIAN_POINT ( 'NONE',  ( -2.452966189433204658, -292.8368583064619202, -337.8648235127503767 ) ) ;
#82324=CARTESIAN_POINT ( 'NONE',  ( -69.28969707544821688, -293.0487016373118081, -204.0546654968482301 ) ) ;
#82325=DIRECTION ( 'NONE',  ( 0.000000000000000000, 0.000000000000000000, 1.000000000000000000 ) ) ;
#82326=CARTESIAN_POINT ( 'NONE',  ( -12.21432891148207212, -293.1903133549178051, -201.5960120414245011 ) ) ;
#82328=CARTESIAN_POINT ( 'NONE',  ( -71.02661073327266195, -281.5145903600248971, -337.7683401800813385 ) ) ;
#82329=CARTESIAN_POINT ( 'NONE',  ( 19.69376410264296240, -294.1959615334767477, -315.9437032427257463 ) ) ;
#82330=CARTESIAN_POINT ( 'NONE',  ( -44.41921528159145538, -283.1392056562684161, -347.0885178160152122 ) ) ;
#82331=CARTESIAN_POINT ( 'NONE',  ( 18.08688398155689825, -282.7594143343150677, -219.0095234404410292 ) ) ;
#82332=CARTESIAN_POINT ( 'NONE',  ( -15.41541560388288268, -285.9950106876013933, -196.5156162487277811 ) ) ;
#82333=CARTESIAN_POINT ( 'NONE',  ( -96.54968594335289822, -289.1805867965553603, -224.5960347188872106 ) ) ;
#82334=CARTESIAN_POINT ( 'NONE',  ( 8.774264289413407525, -280.9125225619765160, -331.1560649499425040 ) ) ;
#82336=CARTESIAN_POINT ( 'NONE',  ( 22.40219264894185258, -285.6417616310222343, -227.4744668200887077 ) ) ;
#82337=CARTESIAN_POINT ( 'NONE',  ( -36.10566880880616480, -287.9573632209215361, -347.0551039967792235 ) ) ;
#82339=CARTESIAN_POINT ( 'NONE',  ( 25.11505198095997926, -295.6905751152608559, -309.7712034197534763 ) ) ;
#82340=CARTESIAN_POINT ( 'NONE',  ( -6.793467250638665078, -278.0842477673292024, -340.4139116144750119 ) ) ;
#82341=CARTESIAN_POINT ( 'NONE',  ( 38.06569873877572263, -291.5719387353748289, -270.3362162858428519 ) ) ;
#82342=CARTESIAN_POINT ( 'NONE',  ( -69.74585591249896765, -279.2800294973382051, -204.9098319310765248 ) ) ;
#82343=CARTESIAN_POINT ( 'NONE',  ( 1.698269939996603028, -292.7254207456073800, -203.9309096179724747 ) ) ;
#82344=CARTESIAN_POINT ( 'NONE',  ( -86.78877972638498761, -283.4509864546686799, -213.1578123247464873 ) ) ;
#82345=CARTESIAN_POINT ( 'NONE',  ( -87.84604204900279001, -279.7582887888356140, -325.8075975232892461 ) ) ;
#82346=CARTESIAN_POINT ( 'NONE',  ( 8.365698332263766801, -293.4677985638718951, -327.6472782796748788 ) ) ;
#82347=CARTESIAN_POINT ( 'NONE',  ( -112.5083667949886461, -270.5523135770945373, -270.3357088371093937 ) ) ;
#82350=CARTESIAN_POINT ( 'NONE',  ( 36.18295524096621563, -283.3658419134645214, -257.4781114522689904 ) ) ;
#82351=CARTESIAN_POINT ( 'NONE',  ( 34.77569810849829679, -292.9044577444097399, -258.5751844807919042 ) ) ;
#82353=CARTESIAN_POINT ( 'NONE',  ( 26.53690525259170840, -296.4086741954485547, -200.3901485728259502 ) ) ;
#82354=CARTESIAN_POINT ( 'NONE',  ( -37.24182466774747979, -297.1121290728679583, -193.5956645125883142 ) ) ;
#82355=CARTESIAN_POINT ( 'NONE',  ( -36.07808213071292158, -290.3518211694541833, -346.8705593816237069 ) ) ;
#82356=CARTESIAN_POINT ( 'NONE',  ( 1.309783167006689730, -288.3533245194732899, -332.2890021995091843 ) ) ;
#82357=CARTESIAN_POINT ( 'NONE',  ( -4.051520344647697058, -282.0194722664597293, -204.6015894868916121 ) ) ;
#82358=CARTESIAN_POINT ( 'NONE',  ( -90.79299233280737269, -299.0416136491614907, -219.0926954798472366 ) ) ;
#82359=CARTESIAN_POINT ( 'NONE',  ( -85.73453516167337796, -278.1592304967379050, -215.1772070919432167 ) ) ;
#82360=ORIENTED_EDGE ( 'NONE', *, *, #27217, .F. ) ;
#82361=CARTESIAN_POINT ( 'NONE',  ( -89.59083614453417965, -297.0064800756047703, -213.7577536588895271 ) ) ;
#82362=CARTESIAN_POINT ( 'NONE',  ( -1.772462948257002679, -294.4473627420438788, -204.9544162125113189 ) ) ;
#82363=CARTESIAN_POINT ( 'NONE',  ( 27.43669690149172524, -295.6836765490610333, -310.5875840072461642 ) ) ;
#82364=CARTESIAN_POINT ( 'NONE',  ( 114.7448031289451222, -299.5541904835127980, -195.3611179825600175 ) ) ;
#82365=CARTESIAN_POINT ( 'NONE',  ( -110.4699854496919329, -291.2285162601526167, -268.4673839537786648 ) ) ;
#82368=CARTESIAN_POINT ( 'NONE',  ( 8.128853119374587877, -290.8056646032590606, -209.6925369026090209 ) ) ;
#82369=CARTESIAN_POINT ( 'NONE',  ( -107.9979751857916312, -272.3074194226331883, -251.5747286257295059 ) ) ;
#82372=CARTESIAN_POINT ( 'NONE',  ( -112.2481029937105603, -292.2567656670873930, -255.7417230204102623 ) ) ;
#82373=CARTESIAN_POINT ( 'NONE',  ( -37.30987171927208124, -297.5519495502701375, -350.3611179825600175 ) ) ;
#82374=CARTESIAN_POINT ( 'NONE',  ( -1.325855163764886324, -288.5307547953036647, -204.7065888023394109 ) ) ;
#82375=CARTESIAN_POINT ( 'NONE',  ( 22.15424010287022938, -272.9291109023894251, -224.9499129657051242 ) ) ;
#82376=CARTESIAN_POINT ( 'NONE',  ( 36.13243484384660320, -277.6309709322517847, -282.6258391460973485 ) ) ;
#82377=CARTESIAN_POINT ( 'NONE',  ( 11.90135421255370041, -290.8220737860941085, -214.4672679067443255 ) ) ;
#82378=CARTESIAN_POINT ( 'NONE',  ( -105.0820021792415702, -280.8575107608771759, -236.3096018622354677 ) ) ;
#82380=CARTESIAN_POINT ( 'NONE',  ( -66.60798983522049355, -282.7944856228870663, -337.3625954408391863 ) ) ;
#82381=CARTESIAN_POINT ( 'NONE',  ( -103.1534298860790102, -280.1484552695858383, -230.8838705315120023 ) ) ;
#82382=CARTESIAN_POINT ( 'NONE',  ( -14.33232856959805979, -279.1388214160971302, -197.2399322328401183 ) ) ;
#82384=CARTESIAN_POINT ( 'NONE',  ( -111.5680120584095363, -268.0791262347229917, -295.3987848039294590 ) ) ;
#82385=CARTESIAN_POINT ( 'NONE',  ( 19.85252384393870884, -275.7961232425344065, -219.0810537184380564 ) ) ;
#82388=CARTESIAN_POINT ( 'NONE',  ( -24.29734724329654583, -275.7357690683512601, -195.1239819704289005 ) ) ;
#82389=CARTESIAN_POINT ( 'NONE',  ( -110.4683760289727132, -299.2662352645559167, -253.7030783399848985 ) ) ;
#82392=CARTESIAN_POINT ( 'NONE',  ( -61.34329307534394360, -290.4510202371023411, -339.6297949535154430 ) ) ;
#82393=CARTESIAN_POINT ( 'NONE',  ( -12.53310460084819233, -290.4941845545233718, -342.2390122968308219 ) ) ;
#82394=CARTESIAN_POINT ( 'NONE',  ( -77.30395300483738197, -290.8490545257827193, -209.1491010820159318 ) ) ;
#82395=CARTESIAN_POINT ( 'NONE',  ( -63.17486536149112197, -285.2321353220696096, -197.8892304868761016 ) ) ;
#82397=CARTESIAN_POINT ( 'NONE',  ( 6.046154686107807485, -280.8522137280722859, -330.0598153541484976 ) ) ;
#82398=CARTESIAN_POINT ( 'NONE',  ( 33.49936643192386043, -289.7037721265573964, -292.7226674005448785 ) ) ;
#82399=CARTESIAN_POINT ( 'NONE',  ( -87.41399834689386239, -282.2453534015842251, -324.5000960783352184 ) ) ;
#82400=CARTESIAN_POINT ( 'NONE',  ( 20.05069849074380173, -282.2231019863413621, -224.4551699962655107 ) ) ;
#82401=CARTESIAN_POINT ( 'NONE',  ( 3.066503686219371527, -289.4652134990666923, -335.6921350426601975 ) ) ;
#82402=CARTESIAN_POINT ( 'NONE',  ( -92.25883456660780269, -279.7318883752008674, -222.1539447692411215 ) ) ;
#82403=CARTESIAN_POINT ( 'NONE',  ( -47.67456082792981675, -290.7186301013121010, -194.4047646367734217 ) ) ;
#82405=CARTESIAN_POINT ( 'NONE',  ( -96.14013522136471579, -284.6872832165995533, -319.8476514505357500 ) ) ;
#82406=CARTESIAN_POINT ( 'NONE',  ( -43.66746537090856606, -286.4667297865374849, -193.6299278297640285 ) ) ;
#82407=CARTESIAN_POINT ( 'NONE',  ( -36.19140285010022495, -283.2040122275516296, -343.3520545480408259 ) ) ;
#82410=CARTESIAN_POINT ( 'NONE',  ( 21.23890289750610094, -294.7567841826703443, -222.3130333863156807 ) ) ;
#82411=CARTESIAN_POINT ( 'NONE',  ( 38.32631535113828392, -292.3791924145763232, -281.6593349319833237 ) ) ;
#82412=CARTESIAN_POINT ( 'NONE',  ( 18.48000754087588149, -275.2828207700454755, -317.7672927031441645 ) ) ;
#82413=CARTESIAN_POINT ( 'NONE',  ( -50.45830788761586660, -294.5638708112776953, -346.1861437054520252 ) ) ;
#82414=CARTESIAN_POINT ( 'NONE',  ( -6.966949695409581977, -290.9380486166039645, -203.2188638474794971 ) ) ;
#82415=CARTESIAN_POINT ( 'NONE',  ( -12.69159266024655786, -292.9672450212768808, -340.2029740491024086 ) ) ;
#82416=CARTESIAN_POINT ( 'NONE',  ( -86.20475253174726049, -292.5617293144588871, -215.5247079408773914 ) ) ;
#82417=CARTESIAN_POINT ( 'NONE',  ( 2.396559803831197932, -293.6777613780329261, -208.6966338344543885 ) ) ;
#82419=CARTESIAN_POINT ( 'NONE',  ( 24.19867358784602374, -292.1369262863266840, -313.5438630105738866 ) ) ;
#82420=CARTESIAN_POINT ( 'NONE',  ( -111.1737870672073996, -298.3821100613930639, -283.6168362630506294 ) ) ;
#82421=CARTESIAN_POINT ( 'NONE',  ( 24.44326591872133747, -289.0353032477154898, -309.6806604337058957 ) ) ;
#82422=CARTESIAN_POINT ( 'NONE',  ( -9.789223836702888093, -278.6739310197044688, -340.4986104771514306 ) ) ;
#82423=CARTESIAN_POINT ( 'NONE',  ( -2.917370278473610412, -275.4023709352172204, -338.8079792516905968 ) ) ;
#82424=CARTESIAN_POINT ( 'NONE',  ( -46.86014843659808804, -273.2828821998430158, -194.0544214992168577 ) ) ;
#82425=CARTESIAN_POINT ( 'NONE',  ( 31.66036271606739660, -279.9987828457924479, -298.2901265364556025 ) ) ;
#82426=CARTESIAN_POINT ( 'NONE',  ( -106.8547622138593880, -276.5477313686046728, -301.7045630273628944 ) ) ;
#82427=CARTESIAN_POINT ( 'NONE',  ( -109.0768573479720374, -295.0276082819629551, -286.3395627853093970 ) ) ;
#82429=CARTESIAN_POINT ( 'NONE',  ( -92.10001089432864774, -273.8945109453640612, -221.9315808135544046 ) ) ;
#82431=CARTESIAN_POINT ( 'NONE',  ( 27.47583976550490092, -286.0839420963176281, -308.7940898036301292 ) ) ;
#82432=CARTESIAN_POINT ( 'NONE',  ( 34.12178154374939254, -275.1881280873132027, -255.4014008279607424 ) ) ;
#82433=CARTESIAN_POINT ( 'NONE',  ( -14.95224843126578662, -288.7700580054889770, -344.0898795096062486 ) ) ;
#82434=CARTESIAN_POINT ( 'NONE',  ( -82.49951617655160874, -275.4376479921858163, -210.2060239856061798 ) ) ;
#82435=CARTESIAN_POINT ( 'NONE',  ( -109.5994094017950289, -294.8033588208400033, -250.8476857577201429 ) ) ;
#82437=CARTESIAN_POINT ( 'NONE',  ( -5.531717702487208399, -281.8414302763886781, -340.3059808331532281 ) ) ;
#82439=CARTESIAN_POINT ( 'NONE',  ( 82.68073018288104947, -297.0543924324409204, -195.4120394483015559 ) ) ;
#82440=CARTESIAN_POINT ( 'NONE',  ( 36.74826726560811352, -279.7056617040976789, -282.3293288460289432 ) ) ;
#82442=CARTESIAN_POINT ( 'NONE',  ( -67.95288029525517004, -290.4360297557573745, -203.6383445090889666 ) ) ;
#82443=CARTESIAN_POINT ( 'NONE',  ( -36.19786556952487189, -281.1772442848348987, -344.5875090164536232 ) ) ;
#82446=CARTESIAN_POINT ( 'NONE',  ( -75.98894803118911057, -289.5362158942540418, -206.0246006044155251 ) ) ;
#82447=CARTESIAN_POINT ( 'NONE',  ( 11.99648687322780560, -276.2726565792751785, -215.5525755127405318 ) ) ;
#82448=CARTESIAN_POINT ( 'NONE',  ( -66.41128102162380742, -284.6294906515863659, -341.2481309384935457 ) ) ;
#82449=CARTESIAN_POINT ( 'NONE',  ( -27.16577893794107013, -272.2602384215733764, -195.4370302956241687 ) ) ;
#82450=CARTESIAN_POINT ( 'NONE',  ( -108.9794944755538069, -284.3669859658438668, -284.3977280088179782 ) ) ;
#82451=CARTESIAN_POINT ( 'NONE',  ( 35.96346016646441512, -276.8856398335441327, -263.3466719203497064 ) ) ;
#82452=CARTESIAN_POINT ( 'NONE',  ( -24.29077734957826351, -277.6842273968209156, -342.4007043862353044 ) ) ;
#82453=CARTESIAN_POINT ( 'NONE',  ( 12.37458611862648716, -284.3604744053404829, -326.5844448629242152 ) ) ;
#82455=CARTESIAN_POINT ( 'NONE',  ( 204.7105398379021040, 292.9631599619078202, -53.99999999999737810 ) ) ;
#82456=CARTESIAN_POINT ( 'NONE',  ( 39.65608403047398411, -293.3489238575383524, -267.4387204345877080 ) ) ;
#82458=CARTESIAN_POINT ( 'NONE',  ( 19.08544293954241766, -290.2386823636759345, -319.7867301798541462 ) ) ;
#82459=CARTESIAN_POINT ( 'NONE',  ( -88.47809603358389552, -288.9094976428775681, -206.1857440867352693 ) ) ;
#82460=CARTESIAN_POINT ( 'NONE',  ( -77.73872415856457962, -276.7767824746940164, -335.7853221518901137 ) ) ;
#82461=CARTESIAN_POINT ( 'NONE',  ( -69.26917854255420082, -290.0389958407305926, -201.1582244431931485 ) ) ;
#82462=CARTESIAN_POINT ( 'NONE',  ( -90.17329783333302373, -286.8088472991352091, -218.9115122137386891 ) ) ;
#82464=CARTESIAN_POINT ( 'NONE',  ( -96.89521200831394765, -279.7044992259339438, -314.3295175566887565 ) ) ;
#82465=CARTESIAN_POINT ( 'NONE',  ( -26.72109892221409666, -287.6098473805943172, -194.6389530431369508 ) ) ;
#82466=CARTESIAN_POINT ( 'NONE',  ( 34.14519963821470583, -283.8470210495419224, -293.2157675015203040 ) ) ;
#82467=CARTESIAN_POINT ( 'NONE',  ( 39.62351893222895427, -275.7648644548721109, -274.0418474908827875 ) ) ;
#82468=CARTESIAN_POINT ( 'NONE',  ( -62.40799748749950027, -277.2026169686447474, -343.2232009398261994 ) ) ;
#82469=CARTESIAN_POINT ( 'NONE',  ( -35.80224228992085500, -299.9917209434586880, -195.9206014286108086 ) ) ;
#82471=CARTESIAN_POINT ( 'NONE',  ( -20.19161114001083490, -279.3376638359844719, -345.3538533559490702 ) ) ;
#82472=CARTESIAN_POINT ( 'NONE',  ( -84.42992257984572291, -295.5513200389712551, -211.0062126747269531 ) ) ;
#82474=CARTESIAN_POINT ( 'NONE',  ( -45.92154307301868954, -276.6713879772625546, -342.9677976229069145 ) ) ;
#82475=CARTESIAN_POINT ( 'NONE',  ( 9.256585017003372329, -275.8815282660360140, -209.5613767083460459 ) ) ;
#82476=CARTESIAN_POINT ( 'NONE',  ( 26.51947287183731916, -281.1733385392578271, -312.9588972198923216 ) ) ;
#82477=CARTESIAN_POINT ( 'NONE',  ( 28.55021068458711042, -288.8592404642445217, -236.5401726730200380 ) ) ;
#82478=CARTESIAN_POINT ( 'NONE',  ( -105.3310694831036898, -297.6207611210693926, -305.1206862837325957 ) ) ;
#82479=CARTESIAN_POINT ( 'NONE',  ( -97.95083187663782098, -297.1286502173527992, -317.2070555743242721 ) ) ;
#82480=CARTESIAN_POINT ( 'NONE',  ( -47.26209866149315530, -293.9259653719904577, -196.1882515306018036 ) ) ;
#82481=CARTESIAN_POINT ( 'NONE',  ( 22.81763154704554708, -278.9430459116272232, -225.8324271297751693 ) ) ;
#82482=CARTESIAN_POINT ( 'NONE',  ( 12.24724870204911120, -282.6689241379756936, -214.8430997424370901 ) ) ;
#82483=CARTESIAN_POINT ( 'NONE',  ( -60.94986093148587969, -295.8233386440902564, -199.7093702652381637 ) ) ;
#82484=CARTESIAN_POINT ( 'NONE',  ( -108.2911461885014575, -286.5099392827481779, -242.4215404325482268 ) ) ;
#82485=CARTESIAN_POINT ( 'NONE',  ( 35.98995588070685159, -286.4456292925386833, -268.3175028324865252 ) ) ;
#82486=CARTESIAN_POINT ( 'NONE',  ( 12.93180314520840390, -280.0814861625955245, -212.1727372273141725 ) ) ;
#82487=CARTESIAN_POINT ( 'NONE',  ( 195.6606144031773624, 277.6437891327478837, -125.5779349732042931 ) ) ;
#82489=CARTESIAN_POINT ( 'NONE',  ( -5.785668917394137800, -286.1455220606764556, -204.4967079756274018 ) ) ;
#82491=CARTESIAN_POINT ( 'NONE',  ( -44.37710816238698897, -284.2187029469874915, -346.7817639628316329 ) ) ;
#82492=CARTESIAN_POINT ( 'NONE',  ( 33.52867671504472469, -275.6533577303742391, -252.7691546761126062 ) ) ;
#82493=CARTESIAN_POINT ( 'NONE',  ( -21.05335969569015475, -285.0516084391568370, -195.5099410818497745 ) ) ;
#82494=CARTESIAN_POINT ( 'NONE',  ( -72.02014421385571552, -290.5248190885428698, -201.9441074920214305 ) ) ;
#82495=CARTESIAN_POINT ( 'NONE',  ( 14.99213384018927897, -281.7097151317625503, -214.1280680830554388 ) ) ;
#82497=CARTESIAN_POINT ( 'NONE',  ( -36.77730032759365031, -281.5792412576677748, -194.0436084626722391 ) ) ;
#82498=CARTESIAN_POINT ( 'NONE',  ( 23.38885489124345796, -282.5177557511680106, -317.6851052038866783 ) ) ;
#82499=CARTESIAN_POINT ( 'NONE',  ( 7.450504543161054372, -290.1952119285918457, -214.2458315076590907 ) ) ;
#82500=CARTESIAN_POINT ( 'NONE',  ( -38.96138201640420107, -140.0153644756211690, -364.8523457303913347 ) ) ;
#82501=VERTEX_POINT ( 'NONE', #32637 ) ;
#82502=CARTESIAN_POINT ( 'NONE',  ( -0.5471318346057595372, -278.5625625246000254, -335.5825473192836625 ) ) ;
#82503=CARTESIAN_POINT ( 'NONE',  ( -40.57655935219229093, -139.1380882315665986, -364.1107628283134545 ) ) ;
#82504=CARTESIAN_POINT ( 'NONE',  ( 32.62056299121131531, -279.2311140906252263, -244.1909987935560480 ) ) ;
#82505=CARTESIAN_POINT ( 'NONE',  ( -70.50638936266145151, -296.9514916630077437, -205.2012279533325625 ) ) ;
#82506=CARTESIAN_POINT ( 'NONE',  ( -30.69633000902539166, -291.6415512030366699, -193.6574660430720769 ) ) ;
#82508=CARTESIAN_POINT ( 'NONE',  ( -34.76575678976643502, -296.6585409844428796, -193.9509524979931996 ) ) ;
#82509=CARTESIAN_POINT ( 'NONE',  ( 31.22093536719553342, -286.3150514432832097, -297.8046255616397389 ) ) ;
#82510=CARTESIAN_POINT ( 'NONE',  ( 2.248281095152399711, -296.3765907232597669, -333.2192939629504167 ) ) ;
#82511=CARTESIAN_POINT ( 'NONE',  ( -70.21796471413269103, -286.9247774450184352, -204.6173688880804207 ) ) ;
#82512=CARTESIAN_POINT ( 'NONE',  ( 32.02256854360830829, -294.9175076157478088, -303.3699990487363607 ) ) ;
#82514=CARTESIAN_POINT ( 'NONE',  ( -101.8225919313987049, -284.5754438083872628, -304.8228607998860298 ) ) ;
#82515=CARTESIAN_POINT ( 'NONE',  ( -101.9731046116610003, -295.8888496526600420, -229.2418977489899135 ) ) ;
#82516=CARTESIAN_POINT ( 'NONE',  ( -74.60954791432716604, -292.3720246158036957, -203.1653864064323614 ) ) ;
#82517=CARTESIAN_POINT ( 'NONE',  ( -69.60308056145483135, -292.1311322703077167, -200.4988796696016209 ) ) ;
#82518=CARTESIAN_POINT ( 'NONE',  ( -95.76704589989074634, -290.1042463191600405, -314.1481634469123492 ) ) ;
#82521=CARTESIAN_POINT ( 'NONE',  ( -43.21797973049908848, -299.8392521455532460, -194.7721816118493052 ) ) ;
#82522=CARTESIAN_POINT ( 'NONE',  ( -100.8706084217704557, -271.9150025699899516, -227.4638311334730076 ) ) ;
#82523=CARTESIAN_POINT ( 'NONE',  ( -7.167449183939760715, -281.7050822454705781, -337.1051002758651407 ) ) ;
#82525=CARTESIAN_POINT ( 'NONE',  ( 19.82727180492823038, -275.7594858833610374, -321.8709823898286686 ) ) ;
#82526=CARTESIAN_POINT ( 'NONE',  ( -46.25542043764335176, -272.3370527488094694, -197.1014018725825849 ) ) ;
#82527=CARTESIAN_POINT ( 'NONE',  ( -84.23605247048401168, -281.2601017368796192, -212.7464547270773778 ) ) ;
#82528=CARTESIAN_POINT ( 'NONE',  ( -24.13270432275103872, -275.0214075023241094, -343.4640216112316011 ) ) ;
#82529=CARTESIAN_POINT ( 'NONE',  ( -110.1966948570239566, -297.6350803071970290, -279.6713539545851859 ) ) ;
#82530=CARTESIAN_POINT ( 'NONE',  ( -40.54518219594275763, -299.0906332331567228, -197.1094297797922650 ) ) ;
#82531=CARTESIAN_POINT ( 'NONE',  ( -99.28325899652840292, -298.7465347038093455, -225.9799992343394877 ) ) ;
#82532=CARTESIAN_POINT ( 'NONE',  ( -68.14807520117722106, -271.6697632744218254, -201.5765881853824908 ) ) ;
#82533=CARTESIAN_POINT ( 'NONE',  ( 19.77860531266616917, -294.8472692415576830, -316.0008455415297703 ) ) ;
#82534=CARTESIAN_POINT ( 'NONE',  ( -25.29489728844791685, -290.7833046504463823, -197.7127380761053814 ) ) ;
#82536=CARTESIAN_POINT ( 'NONE',  ( 37.57355239530809854, -275.8244566266408810, -252.7757981883405023 ) ) ;
#82537=CARTESIAN_POINT ( 'NONE',  ( -87.33484883728418424, -273.4984532070666887, -217.0971217899188446 ) ) ;
#82538=CARTESIAN_POINT ( 'NONE',  ( 29.32391031239793477, -280.7283780216035893, -308.0056250998787846 ) ) ;
#82540=CARTESIAN_POINT ( 'NONE',  ( -110.2575368903987254, -283.6704687388914294, -276.3513163007959861 ) ) ;
#82541=CARTESIAN_POINT ( 'NONE',  ( -89.19237935618261304, -281.7789361055441759, -324.8525023825768017 ) ) ;
#82542=CARTESIAN_POINT ( 'NONE',  ( 34.95575594754692617, -273.9472338617135279, -256.6333081294811223 ) ) ;
#82543=CARTESIAN_POINT ( 'NONE',  ( -18.37500761558206008, -282.2965549838534685, -197.7458778143534346 ) ) ;
#82546=CARTESIAN_POINT ( 'NONE',  ( 121.3395553409046670, -299.5541904835127980, -195.3611179825600175 ) ) ;
#82547=CARTESIAN_POINT ( 'NONE',  ( 4.441702967271813129, -273.0051304735683857, -206.5757633865261482 ) ) ;
#82548=CARTESIAN_POINT ( 'NONE',  ( -98.15124213503874273, -279.9515046995883267, -314.5670193432101769 ) ) ;
#82551=CARTESIAN_POINT ( 'NONE',  ( -78.35716676517075996, -285.5195928006980921, -333.8201259565773285 ) ) ;
#82554=CARTESIAN_POINT ( 'NONE',  ( -108.6127905447404061, -288.8555574166600763, -246.8444638832748126 ) ) ;
#82556=CARTESIAN_POINT ( 'NONE',  ( -94.75236337395298847, -295.9893873475351143, -224.6320653799195100 ) ) ;
#82557=CARTESIAN_POINT ( 'NONE',  ( -89.54625175619254662, -287.9371772843049939, -323.1394304648690650 ) ) ;
#82559=CARTESIAN_POINT ( 'NONE',  ( -94.24566304080687473, -295.2291774487622433, -221.4850559888845396 ) ) ;
#82560=CARTESIAN_POINT ( 'NONE',  ( 25.27160399030096016, -286.6147049481688214, -314.0669675456417167 ) ) ;
#82561=CARTESIAN_POINT ( 'NONE',  ( 33.88033775284389293, -282.8990588323061388, -250.9773150130828583 ) ) ;
#82562=CARTESIAN_POINT ( 'NONE',  ( -93.66333683618501027, -282.0897228687630331, -321.3887287345775690 ) ) ;
#82563=CARTESIAN_POINT ( 'NONE',  ( 3.614607755860435478, -288.4844018644666335, -330.8503828652974903 ) ) ;
#82564=CARTESIAN_POINT ( 'NONE',  ( 26.07596077042461147, -283.4872486566332555, -307.7924733455990349 ) ) ;
#82565=CARTESIAN_POINT ( 'NONE',  ( 35.84866676538538854, -282.3314068456118662, -268.5694435731335261 ) ) ;
#82566=CARTESIAN_POINT ( 'NONE',  ( 35.91158350479658168, -289.7585610763740647, -288.0895074394872495 ) ) ;
#82567=CARTESIAN_POINT ( 'NONE',  ( -78.20426114684735808, -297.6853195782457533, -205.0981797136934688 ) ) ;
#82568=CARTESIAN_POINT ( 'NONE',  ( -63.55709447827728553, -273.7197109947475155, -197.9611656409754517 ) ) ;
#82569=CARTESIAN_POINT ( 'NONE',  ( 14.01698657334408971, -294.7572256928926322, -216.1934883399696616 ) ) ;
#82571=CARTESIAN_POINT ( 'NONE',  ( 31.98288692825981272, -284.4805209788416960, -303.7098442033569654 ) ) ;
#82573=CARTESIAN_POINT ( 'NONE',  ( 36.10863148312927962, -273.7573775827134455, -286.3922995662848052 ) ) ;
#82575=CARTESIAN_POINT ( 'NONE',  ( -112.8066049457675746, -295.0866563836123078, -259.7080953377011383 ) ) ;
#82576=CARTESIAN_POINT ( 'NONE',  ( -102.3381664136654905, -291.6794734305941574, -305.4250944542794173 ) ) ;
#82577=CARTESIAN_POINT ( 'NONE',  ( 7.399835882282070010, -274.0295742914274228, -212.5503264012068314 ) ) ;
#82578=CARTESIAN_POINT ( 'NONE',  ( -97.10970357946827392, -291.4750224174902087, -313.4713663806534214 ) ) ;
#82579=CARTESIAN_POINT ( 'NONE',  ( -38.91461170556577542, -292.9731931671891516, -197.1427159379056491 ) ) ;
#82580=CARTESIAN_POINT ( 'NONE',  ( -74.28339403856894307, -285.3101900770944894, -334.5544118177253381 ) ) ;
#82581=CARTESIAN_POINT ( 'NONE',  ( -112.3500599257388473, -292.1619313333140440, -255.7205636520275505 ) ) ;
#82582=CARTESIAN_POINT ( 'NONE',  ( -98.81838416704960082, -292.4768482241271386, -224.7989022750655579 ) ) ;
#82583=CARTESIAN_POINT ( 'NONE',  ( 27.15707567323472560, -293.8525071746819322, -304.6584254100509384 ) ) ;
#82584=CARTESIAN_POINT ( 'NONE',  ( 35.65334380386608615, -289.7734966758292785, -287.5868027192905743 ) ) ;
#82585=CARTESIAN_POINT ( 'NONE',  ( 24.59047896289302315, -281.1107767252492522, -224.6073728072628626 ) ) ;
#82586=CARTESIAN_POINT ( 'NONE',  ( -112.8977929396748152, -294.6417942402715653, -269.5923304998602248 ) ) ;
#82587=CARTESIAN_POINT ( 'NONE',  ( -63.91400756646391557, -283.2226280652972719, -342.6308383494057921 ) ) ;
#82588=CARTESIAN_POINT ( 'NONE',  ( 37.01431119181969365, -277.4401703778087835, -263.2392892275520921 ) ) ;
#82589=CARTESIAN_POINT ( 'NONE',  ( -1.891800215404187080, -284.5216069148665952, -204.2679621557210226 ) ) ;
#82590=CARTESIAN_POINT ( 'NONE',  ( -17.70129934298482510, -274.9410343472310956, -343.5359779752348572 ) ) ;
#82592=CARTESIAN_POINT ( 'NONE',  ( 7.827089652886396465, -281.9239375541179129, -327.8519300419252431 ) ) ;
#82593=CARTESIAN_POINT ( 'NONE',  ( -97.39522090471874094, -280.3968677798985709, -222.8050104575527541 ) ) ;
#82594=CARTESIAN_POINT ( 'NONE',  ( 11.93574416855805964, -285.7761448799196842, -211.4312863813052275 ) ) ;
#82595=CARTESIAN_POINT ( 'NONE',  ( -38.33369865619360439, -296.8248972015235267, -344.3678065667407964 ) ) ;
#82596=CARTESIAN_POINT ( 'NONE',  ( 25.41968024469691656, -277.7297915252465828, -313.6664750327792035 ) ) ;
#82597=CARTESIAN_POINT ( 'NONE',  ( 39.06077961077273386, -276.8055662932858922, -265.4546053573145628 ) ) ;
#82598=CARTESIAN_POINT ( 'NONE',  ( -109.0436849915936932, -278.2038091855637276, -284.1321152679568058 ) ) ;
#82599=CARTESIAN_POINT ( 'NONE',  ( -37.86015303360545659, -300.0458004339149056, -195.5295762530892603 ) ) ;
#82600=CARTESIAN_POINT ( 'NONE',  ( -8.770429384935741979, -284.4266351339829839, -201.1828923952035950 ) ) ;
#82601=CARTESIAN_POINT ( 'NONE',  ( 39.21557064413320859, -293.3256510229967375, -278.8967413848646970 ) ) ;
#82602=CARTESIAN_POINT ( 'NONE',  ( -80.07494018488009146, -291.2197485293272052, -333.5145528107659061 ) ) ;
#82603=CARTESIAN_POINT ( 'NONE',  ( -32.12160937787644599, -291.0398354033779924, -197.2254196230580874 ) ) ;
#82605=CARTESIAN_POINT ( 'NONE',  ( 30.84965138493864956, -292.8701859719204776, -244.2454700766830911 ) ) ;
#82607=CARTESIAN_POINT ( 'NONE',  ( -69.21623923897220720, -290.5413702480978486, -340.1286633109422155 ) ) ;
#82608=CARTESIAN_POINT ( 'NONE',  ( -34.31740431005579950, -280.7425553907566496, -197.3092092615671049 ) ) ;
#82609=CARTESIAN_POINT ( 'NONE',  ( -70.58257500928206696, -296.5443779058055043, -201.2486245488751706 ) ) ;
#82610=CARTESIAN_POINT ( 'NONE',  ( 23.77536475374988001, -287.5802677178115232, -223.6702998242654417 ) ) ;
#82611=CARTESIAN_POINT ( 'NONE',  ( 38.65479868520689166, -288.0428418929850523, -282.9440296418400180 ) ) ;
#82612=CARTESIAN_POINT ( 'NONE',  ( -97.54737581831494708, -284.3093522370493247, -311.7694993780186223 ) ) ;
#82613=CARTESIAN_POINT ( 'NONE',  ( -108.0627147292182570, -262.2579186427456648, -317.5738021120234862 ) ) ;
#82614=CARTESIAN_POINT ( 'NONE',  ( 195.4949434911534922, 284.6999941648707022, -111.1574007831435154 ) ) ;
#82615=CARTESIAN_POINT ( 'NONE',  ( -63.17214948145560527, -182.5205970719807738, -358.6122145540047086 ) ) ;
#82616=CARTESIAN_POINT ( 'NONE',  ( -87.21305541279318163, -276.9660883578187622, -323.8910128888574604 ) ) ;
#82617=CARTESIAN_POINT ( 'NONE',  ( 22.71118079196729411, -275.0574298264636468, -312.4943834877149129 ) ) ;
#82618=CARTESIAN_POINT ( 'NONE',  ( -70.11890833012333246, -273.2988161754577732, -200.6947246028664438 ) ) ;
#82619=CARTESIAN_POINT ( 'NONE',  ( -11.41673792228423601, -92.95531928750351369, -356.8092562351845345 ) ) ;
#82620=CARTESIAN_POINT ( 'NONE',  ( -5.505355017525573658, -275.3268730155184585, -339.9293967055468215 ) ) ;
#82622=CARTESIAN_POINT ( 'NONE',  ( -53.41597137761358027, -289.7563088466230852, -341.6324743976787772 ) ) ;
#82623=CARTESIAN_POINT ( 'NONE',  ( -103.7154863750676697, -297.8609436063642306, -231.5434584901159667 ) ) ;
#82624=CARTESIAN_POINT ( 'NONE',  ( -110.2853717116281445, -296.7361208981710092, -294.8304391642227529 ) ) ;
#82625=CARTESIAN_POINT ( 'NONE',  ( -39.68691106817787784, -295.2490684964203069, -343.3358674342650829 ) ) ;
#82627=CARTESIAN_POINT ( 'NONE',  ( -99.27099385811067123, -279.8890961074330335, -313.6517263983822090 ) ) ;
#82628=CARTESIAN_POINT ( 'NONE',  ( 39.64889698460557810, -281.0544958251629168, -269.9368704188668175 ) ) ;
#82629=CARTESIAN_POINT ( 'NONE',  ( -108.1151075438105948, -279.3804103635697516, -289.4752718236618421 ) ) ;
#82630=CARTESIAN_POINT ( 'NONE',  ( -23.10646233388825266, -278.6327681548443707, -345.0559482293683686 ) ) ;
#82631=CARTESIAN_POINT ( 'NONE',  ( -96.56380144823381784, -295.7344619146651326, -226.6578447667980640 ) ) ;
#82633=CARTESIAN_POINT ( 'NONE',  ( -102.1568603758254312, -279.1769078233310211, -236.6654606890924697 ) ) ;
#82634=CARTESIAN_POINT ( 'NONE',  ( -94.03305062971648454, -274.0620831594770266, -218.4740720280185542 ) ) ;
#82635=CARTESIAN_POINT ( 'NONE',  ( -51.60985992745454354, -287.9158295728792609, -345.5257232660986801 ) ) ;
#82636=CARTESIAN_POINT ( 'NONE',  ( -11.07262430503478967, -276.3945657468199784, -200.0567740324949852 ) ) ;
#82637=CARTESIAN_POINT ( 'NONE',  ( 37.60089007749757428, -274.3147539457711446, -285.2679777379279926 ) ) ;
#82639=CARTESIAN_POINT ( 'NONE',  ( -107.1091775830442003, -289.4560039153885782, -292.5537591798423591 ) ) ;
#82640=CARTESIAN_POINT ( 'NONE',  ( -87.67694735806045969, -284.7195231201136494, -212.1556522290955229 ) ) ;
#82642=CARTESIAN_POINT ( 'NONE',  ( 12.58394688920153826, -280.5845251003603948, -324.9999666293288669 ) ) ;
#82643=CARTESIAN_POINT ( 'NONE',  ( 30.87399498264696973, -280.4935849232745682, -297.9653541863594910 ) ) ;
#82644=CARTESIAN_POINT ( 'NONE',  ( -97.72894036780775195, -283.2292077500413825, -226.8112825950305478 ) ) ;
#82645=CARTESIAN_POINT ( 'NONE',  ( -24.29099974948256957, -290.8858280170737771, -344.2688895372364186 ) ) ;
#82646=CARTESIAN_POINT ( 'NONE',  ( -109.4303925683215652, -279.5753431878352444, -284.2242261654769777 ) ) ;
#82647=CARTESIAN_POINT ( 'NONE',  ( -104.5910534586188589, -255.9060656293385989, -326.6254513314219139 ) ) ;
#82648=CARTESIAN_POINT ( 'NONE',  ( -38.73852839177641982, -281.4692759706787228, -346.5483169648414901 ) ) ;
#82649=CARTESIAN_POINT ( 'NONE',  ( -17.02356063911942030, -296.7901157087697470, -342.6103087162557017 ) ) ;
#82650=CARTESIAN_POINT ( 'NONE',  ( -107.5674965909905012, -277.1658173271779901, -241.3385143299554727 ) ) ;
#82651=CARTESIAN_POINT ( 'NONE',  ( -69.65825519134533295, -285.4766550003523093, -338.2403106449377788 ) ) ;
#82653=CARTESIAN_POINT ( 'NONE',  ( -37.47405358822830124, -290.9739089115015531, -345.9338338305279308 ) ) ;
#82654=CARTESIAN_POINT ( 'NONE',  ( 38.39942985181230029, -286.5861810557560148, -257.3437913080956605 ) ) ;
#82655=CARTESIAN_POINT ( 'NONE',  ( -111.0433154238982780, -289.0132993949669071, -265.6646214354952349 ) ) ;
#82657=CARTESIAN_POINT ( 'NONE',  ( 35.84357901833165272, -274.3250249106911838, -277.0811175013301408 ) ) ;
#82658=CARTESIAN_POINT ( 'NONE',  ( 19.76843211831537772, -292.3532529700270857, -317.7878855092637878 ) ) ;
#82661=CARTESIAN_POINT ( 'NONE',  ( 37.67206707051568770, -292.2094440787570875, -284.4188511318005226 ) ) ;
#82662=CARTESIAN_POINT ( 'NONE',  ( -33.21407053015408906, -287.7049835599435710, -196.6262679367014812 ) ) ;
#82663=CARTESIAN_POINT ( 'NONE',  ( -84.55285909274054745, -287.9316533694936879, -329.9688450384134057 ) ) ;
#82664=EDGE_CURVE ( 'NONE', #11917, #37641, #80716, .T. ) ;
#82665=CARTESIAN_POINT ( 'NONE',  ( -14.39939831981606844, -287.7806520233210676, -200.3861085171127741 ) ) ;
#82667=CARTESIAN_POINT ( 'NONE',  ( 18.77906285491499716, -287.6900201410286400, -223.4048200442942971 ) ) ;
#82668=CARTESIAN_POINT ( 'NONE',  ( 19.12900634803856192, -294.8414104928188522, -220.4470812307741028 ) ) ;
#82670=CARTESIAN_POINT ( 'NONE',  ( 34.47660204158474784, -288.4185554214476497, -243.7126622799101483 ) ) ;
#82671=CARTESIAN_POINT ( 'NONE',  ( -111.0844966203669770, -276.4220775833927064, -286.8327350287990498 ) ) ;
#82672=CARTESIAN_POINT ( 'NONE',  ( -45.64311740325929634, -277.4877798357739493, -346.9440955677438865 ) ) ;
#82673=CARTESIAN_POINT ( 'NONE',  ( -6.452805671416432354, -290.5344860512749392, -201.3892056776026322 ) ) ;
#82674=CARTESIAN_POINT ( 'NONE',  ( -100.2489854180985134, -279.1397015698619271, -225.9575881967378450 ) ) ;
#82675=CARTESIAN_POINT ( 'NONE',  ( -93.08972448126661448, -299.2261675601404249, -220.7223772155265920 ) ) ;
#82677=CARTESIAN_POINT ( 'NONE',  ( -82.66756569741487226, -283.4324854704220229, -210.6069000886882918 ) ) ;
#82679=CARTESIAN_POINT ( 'NONE',  ( -95.43420940212885739, -276.0497198911135115, -316.5996718223453286 ) ) ;
#82680=CARTESIAN_POINT ( 'NONE',  ( 34.27374110199472312, -279.2646916449808145, -248.0849148375886557 ) ) ;
#82682=CARTESIAN_POINT ( 'NONE',  ( 7.815040061342853228, -274.9281341120441766, -331.9373103461265941 ) ) ;
#82683=CARTESIAN_POINT ( 'NONE',  ( -108.9683648724278129, -297.8451196095738851, -287.7442685108308069 ) ) ;
#82684=CARTESIAN_POINT ( 'NONE',  ( -58.41506468419694187, -282.2385559931179273, -344.1551638674872038 ) ) ;
#82685=CARTESIAN_POINT ( 'NONE',  ( -106.0306805115512532, -297.8327591180453169, -244.8133516173032547 ) ) ;
#82686=CARTESIAN_POINT ( 'NONE',  ( -112.4081001270483853, -298.0541567665791831, -255.5175469707473610 ) ) ;
#82687=CARTESIAN_POINT ( 'NONE',  ( -2.899937073685689093, -274.1874127323891912, -205.9728236695579540 ) ) ;
#82688=CARTESIAN_POINT ( 'NONE',  ( 27.53513763808576797, -296.0547708550434436, -307.9908478255579212 ) ) ;
#82689=CARTESIAN_POINT ( 'NONE',  ( 23.28877289939664763, -288.3534731135702032, -317.8475547658508162 ) ) ;
#82690=CARTESIAN_POINT ( 'NONE',  ( -111.8130237502571589, -276.7948821461369562, -257.5808144914827267 ) ) ;
#82691=CARTESIAN_POINT ( 'NONE',  ( -114.1877049332714336, -290.4463460359769442, -265.4937213509765570 ) ) ;
#82692=CARTESIAN_POINT ( 'NONE',  ( 27.23229400141799772, -287.0816336101535171, -305.0176455083908422 ) ) ;
#82693=CARTESIAN_POINT ( 'NONE',  ( -78.47566196037180930, -289.4987559711255471, -207.5854330217459562 ) ) ;
#82696=CARTESIAN_POINT ( 'NONE',  ( 33.13960303141829655, -287.3160736852578339, -289.7939093406765778 ) ) ;
#82698=CARTESIAN_POINT ( 'NONE',  ( -104.2061576972415651, -285.0013527830554381, -308.1776965268672939 ) ) ;
#82699=CARTESIAN_POINT ( 'NONE',  ( -34.95568146608258786, -291.1401528551502906, -193.6203917491107518 ) ) ;
#82700=CARTESIAN_POINT ( 'NONE',  ( 21.34144319582575733, -282.4919482016939014, -221.7532059971955221 ) ) ;
#82701=CARTESIAN_POINT ( 'NONE',  ( 20.68108636255614741, -282.1896745242881366, -220.4748362914795621 ) ) ;
#82702=CARTESIAN_POINT ( 'NONE',  ( -40.23648350190087086, -282.9228696131830247, -343.3036997420605871 ) ) ;
#82703=CARTESIAN_POINT ( 'NONE',  ( -112.2743570698698932, -296.7738131870418101, -252.6383381880629031 ) ) ;
#82704=CARTESIAN_POINT ( 'NONE',  ( -72.15602567404700096, -274.8970573560998787, -205.5803303280068235 ) ) ;
#82705=CARTESIAN_POINT ( 'NONE',  ( -55.38609741380400209, -289.8389449761008905, -197.9301403126762295 ) ) ;
#82706=CARTESIAN_POINT ( 'NONE',  ( -34.45088070096986854, -297.0095029632991555, -197.0525493443111316 ) ) ;
#82709=CARTESIAN_POINT ( 'NONE',  ( -70.84148295216125746, -285.4176892182586016, -336.8515221404543922 ) ) ;
#82710=CARTESIAN_POINT ( 'NONE',  ( -55.98179343265648811, -296.3664392228982365, -344.7522426580285355 ) ) ;
#82711=CARTESIAN_POINT ( 'NONE',  ( -108.1294409584828600, -285.4441195427221487, -252.1131477773129745 ) ) ;
#82712=CARTESIAN_POINT ( 'NONE',  ( 37.36011244662669384, -274.8333051002460365, -288.0942205086595322 ) ) ;
#82713=CARTESIAN_POINT ( 'NONE',  ( -0.8595405818749501936, -293.1750667910442871, -202.6679512547323156 ) ) ;
#82714=CARTESIAN_POINT ( 'NONE',  ( 32.72629322408224084, -285.3179313603616265, -241.4006673775781451 ) ) ;
#82715=CARTESIAN_POINT ( 'NONE',  ( -70.89233285013889940, -291.9548175736801454, -201.0783687903830810 ) ) ;
#82716=CARTESIAN_POINT ( 'NONE',  ( -90.60527286799126045, -290.1661487132856792, -320.3857224790692158 ) ) ;
#82718=CARTESIAN_POINT ( 'NONE',  ( 193.4945526529483004, 275.6671624809070522, -124.0448087994775506 ) ) ;
#82719=CARTESIAN_POINT ( 'NONE',  ( -97.05009447858296312, -286.7141478988249332, -222.8467475244120521 ) ) ;
#82720=CARTESIAN_POINT ( 'NONE',  ( -117.3417001280813423, -270.0523547857346784, -270.3292895737509980 ) ) ;
#82722=CARTESIAN_POINT ( 'NONE',  ( -33.49369145353480093, -281.9229382103779926, -343.5817960136208171 ) ) ;
#82723=CARTESIAN_POINT ( 'NONE',  ( -100.2292613782641268, -278.8064742117943524, -225.9663104984124402 ) ) ;
#82724=CARTESIAN_POINT ( 'NONE',  ( -66.81463839377062186, -281.6652702852802008, -201.5621477225321030 ) ) ;
#82725=CARTESIAN_POINT ( 'NONE',  ( -87.50854530310770940, -231.0822326819537125, -346.2094061126495035 ) ) ;
#82726=CARTESIAN_POINT ( 'NONE',  ( 19.33417293193931386, -280.8288916774297945, -321.6874255993433849 ) ) ;
#82727=CARTESIAN_POINT ( 'NONE',  ( 12.24512182097605439, -284.7659169116992643, -214.4974397944724274 ) ) ;
#82728=CARTESIAN_POINT ( 'NONE',  ( -36.57621667797722864, -299.8217447531536664, -194.3742189733497412 ) ) ;
#82729=CARTESIAN_POINT ( 'NONE',  ( -15.56851597490403094, -295.2551345107175393, -340.1561228152332319 ) ) ;
#82731=CARTESIAN_POINT ( 'NONE',  ( 31.29489413764245143, -291.8884512872410824, -244.0882916261481910 ) ) ;
#82732=CARTESIAN_POINT ( 'NONE',  ( -20.14082370990913518, -277.4882817183074621, -345.3653664877197116 ) ) ;
#82733=CARTESIAN_POINT ( 'NONE',  ( 17.28555423567391003, -274.8595207988013840, -221.8624298593667845 ) ) ;
#82734=CARTESIAN_POINT ( 'NONE',  ( 18.66802608855529755, -275.1899028931458133, -322.7481686620251935 ) ) ;
#82736=CARTESIAN_POINT ( 'NONE',  ( -92.87566169342767353, -271.2553444005300776, -219.9341805632221565 ) ) ;
#82737=CARTESIAN_POINT ( 'NONE',  ( 23.57033717333462519, -295.5967514715791253, -316.4949451208443634 ) ) ;
#82740=CARTESIAN_POINT ( 'NONE',  ( -85.05258610946458475, -284.8088302575832813, -326.0198767863370790 ) ) ;
#82741=CARTESIAN_POINT ( 'NONE',  ( 31.09889243830337335, -282.8817270379560114, -237.2271233592184103 ) ) ;
#82742=CARTESIAN_POINT ( 'NONE',  ( -109.6004073896432089, -283.7506106202282012, -281.7573351787241904 ) ) ;
#82743=CARTESIAN_POINT ( 'NONE',  ( -72.04823335984063704, -275.9189552488670643, -335.5052208242718166 ) ) ;
#82744=CARTESIAN_POINT ( 'NONE',  ( -13.10406117072809629, -284.5944561863594799, -340.5825965516420979 ) ) ;
#82745=CARTESIAN_POINT ( 'NONE',  ( -110.9736808483926751, -276.9927348496441368, -273.3676385437074714 ) ) ;
#82746=CARTESIAN_POINT ( 'NONE',  ( 15.66081065149025520, -275.9036331025588993, -219.6422165792442343 ) ) ;
#82748=CARTESIAN_POINT ( 'NONE',  ( -42.42959129426654385, -280.7923453722279419, -193.6912269948513483 ) ) ;
#82752=CARTESIAN_POINT ( 'NONE',  ( -84.75860719134092847, -287.2668094311005120, -211.2684585202955247 ) ) ;
#82753=CARTESIAN_POINT ( 'NONE',  ( -67.37081589559861072, -294.6535087023048618, -337.0895759557257634 ) ) ;
#82754=CARTESIAN_POINT ( 'NONE',  ( -108.7069508600283427, -289.5367807159792051, -299.0022383218778259 ) ) ;
#82756=CARTESIAN_POINT ( 'NONE',  ( -6.575102009894068900, -284.7016297095457844, -203.0315949599066698 ) ) ;
#82757=CARTESIAN_POINT ( 'NONE',  ( -1.886686672506649787, -285.1058752426429237, -205.8189243368559289 ) ) ;
#82758=CARTESIAN_POINT ( 'NONE',  ( -107.9618679548543412, -289.0820992842319015, -248.1652288727090081 ) ) ;
#82760=CARTESIAN_POINT ( 'NONE',  ( -99.95603228407691176, -286.2832018467763078, -231.9683527268942953 ) ) ;
#82761=CARTESIAN_POINT ( 'NONE',  ( -111.7844347963764164, -276.4295217774460980, -279.8992098705120952 ) ) ;
#82762=CARTESIAN_POINT ( 'NONE',  ( -34.71501785021659003, -287.4195387998131537, -346.5158352187889932 ) ) ;
#82763=CARTESIAN_POINT ( 'NONE',  ( -59.93241545100775625, -287.7597293104752225, -198.7901258682998105 ) ) ;
#82764=CARTESIAN_POINT ( 'NONE',  ( 35.71634548336695048, -285.7791524837772954, -288.0945093259146006 ) ) ;
#82765=CARTESIAN_POINT ( 'NONE',  ( -42.93897668876243756, -284.0656428959548521, -343.4324517478227108 ) ) ;
#82766=CARTESIAN_POINT ( 'NONE',  ( 21.85966918795955394, -290.1866567733507054, -316.6984390386710970 ) ) ;
#82769=CARTESIAN_POINT ( 'NONE',  ( -86.54348102956033983, -299.2954201383030863, -212.9466892647377847 ) ) ;
#82770=CARTESIAN_POINT ( 'NONE',  ( 20.39153895366267477, -278.8910007581684454, -222.4676585399201656 ) ) ;
#82771=CARTESIAN_POINT ( 'NONE',  ( -66.94377033987781545, -290.8710914066187456, -199.4535989180087370 ) ) ;
#82772=CARTESIAN_POINT ( 'NONE',  ( -92.42861545285818181, -295.6467252407230148, -221.2503027160147440 ) ) ;
#82773=CARTESIAN_POINT ( 'NONE',  ( 34.96766585705044861, -280.4100423591858089, -283.5692441020132151 ) ) ;
#82774=CARTESIAN_POINT ( 'NONE',  ( 23.47107851813291646, -273.0441217582940112, -227.4074676085840849 ) ) ;
#82775=CARTESIAN_POINT ( 'NONE',  ( -18.07520203310480866, -296.1137166878982043, -341.2839318569509715 ) ) ;
#82776=CARTESIAN_POINT ( 'NONE',  ( -36.17789667918795260, -296.5463577611643586, -194.0547409687907816 ) ) ;
#82777=CARTESIAN_POINT ( 'NONE',  ( 37.35691069979294809, -291.9694636143319144, -284.3629889643822253 ) ) ;
#82778=ADVANCED_FACE ( 'NONE', ( #76649 ), #67150, .F. ) ;
#82779=CARTESIAN_POINT ( 'NONE',  ( 31.37215227949393537, -294.6284562002351208, -244.0213874712032123 ) ) ;
#82781=CARTESIAN_POINT ( 'NONE',  ( 19.46471694001170860, -293.7039029141920992, -224.2367232595827033 ) ) ;
#82783=CARTESIAN_POINT ( 'NONE',  ( -64.67949926195328203, -281.4274201874051187, -340.5964669230062896 ) ) ;
#82784=CARTESIAN_POINT ( 'NONE',  ( -58.40823811073137506, -295.3322039903329141, -340.2553307431710437 ) ) ;
#82785=CARTESIAN_POINT ( 'NONE',  ( -47.25636174880325768, -283.1748236534072589, -346.7201350332435936 ) ) ;
#82786=CARTESIAN_POINT ( 'NONE',  ( -1.834159632218011149, -282.4389747927017993, -203.6638259229042944 ) ) ;
#82787=CARTESIAN_POINT ( 'NONE',  ( -111.6996801312540981, -284.4705698404659415, -250.2451169168295451 ) ) ;
#82788=CARTESIAN_POINT ( 'NONE',  ( -109.5002789043550138, -288.2942020714835394, -290.3807832907983766 ) ) ;
#82790=CARTESIAN_POINT ( 'NONE',  ( 37.73986327910122895, -280.2048168028057944, -284.0522067300307185 ) ) ;
#82791=CARTESIAN_POINT ( 'NONE',  ( 21.24395799978772814, -287.1419309063351193, -319.8506438687795708 ) ) ;
#82793=CARTESIAN_POINT ( 'NONE',  ( -0.3393806837994166603, -296.1519040673607606, -334.2729459834377508 ) ) ;
#82794=CARTESIAN_POINT ( 'NONE',  ( -8.093261221506073966, -278.1017688909275307, -340.9666196044255457 ) ) ;
#82795=CARTESIAN_POINT ( 'NONE',  ( -11.73175743242412317, -280.0615956521529029, -201.9247634153635431 ) ) ;
#82796=CARTESIAN_POINT ( 'NONE',  ( 32.18505200082140760, -293.2932708431480364, -237.1459647922381748 ) ) ;
#82797=CARTESIAN_POINT ( 'NONE',  ( -67.89562980136560100, -283.7341030547903529, -201.2400554045759691 ) ) ;
#82798=ADVANCED_FACE ( 'NONE', ( #11774, #48684 ), #25064, .F. ) ;
#82799=CARTESIAN_POINT ( 'NONE',  ( -98.81132755655988831, -279.9690896055897724, -313.3318702873985444 ) ) ;
#82800=CARTESIAN_POINT ( 'NONE',  ( 35.14232812948045392, -292.4733153081567139, -259.8981310393356239 ) ) ;
#82801=CARTESIAN_POINT ( 'NONE',  ( 6.552430141662815899, -296.6014479846594440, -195.3760751224127148 ) ) ;
#82804=CARTESIAN_POINT ( 'NONE',  ( 20.56814955047110516, -293.6864495690679178, -314.9286281643392726 ) ) ;
#82806=CARTESIAN_POINT ( 'NONE',  ( -67.74223827176246004, -286.9809262143061233, -333.4151289067050357 ) ) ;
#82807=CARTESIAN_POINT ( 'NONE',  ( 75.96719185516560913, -298.4969465617371043, -193.6139409516525234 ) ) ;
#82808=CARTESIAN_POINT ( 'NONE',  ( -63.05157882450594542, -287.0393651260587831, -198.3034993037626350 ) ) ;
#82809=CARTESIAN_POINT ( 'NONE',  ( 10.11365232749199983, -288.2099638290789585, -325.8985728698052071 ) ) ;
#82810=CARTESIAN_POINT ( 'NONE',  ( -110.9720947877023605, -280.0324894246721783, -273.4062342281841325 ) ) ;
#82811=CARTESIAN_POINT ( 'NONE',  ( -104.6493277493149634, -298.7232165756729501, -239.4536348703825013 ) ) ;
#82812=CARTESIAN_POINT ( 'NONE',  ( -104.8010204009342772, -277.7334801601004415, -241.4410451597475458 ) ) ;
#82814=CARTESIAN_POINT ( 'NONE',  ( -95.55232274525623382, -296.9001860716596184, -219.9102700484123432 ) ) ;
#82815=CARTESIAN_POINT ( 'NONE',  ( -106.0412880239350102, -292.8509435957824394, -241.5618981299570862 ) ) ;
#82816=CARTESIAN_POINT ( 'NONE',  ( 37.27433847888814711, -294.9561397021130915, -254.8412711491692733 ) ) ;
#82818=CARTESIAN_POINT ( 'NONE',  ( -103.6522603921755632, -291.6183337501316259, -239.5909658007630867 ) ) ;
#82820=CARTESIAN_POINT ( 'NONE',  ( -37.76398388588894051, -290.1865063346749594, -194.5974910816274814 ) ) ;
#82821=CARTESIAN_POINT ( 'NONE',  ( -114.2801616667020568, -273.0444201233731860, -270.3673729185637171 ) ) ;
#82822=CARTESIAN_POINT ( 'NONE',  ( 8.949707485552313102, -298.3140883898317384, -197.3426842153452867 ) ) ;
#82825=CARTESIAN_POINT ( 'NONE',  ( -84.71891230408671447, -291.2113887296227972, -330.2458053272778784 ) ) ;
#82826=CARTESIAN_POINT ( 'NONE',  ( -72.02372285203398405, -291.9805209788416391, -342.4524372437778652 ) ) ;
#82827=CARTESIAN_POINT ( 'NONE',  ( -68.32954631163414660, -287.6443072018306566, -202.2451740420654858 ) ) ;
#82828=CARTESIAN_POINT ( 'NONE',  ( -16.09638144493141709, -272.3271897830597936, -198.5528820329859343 ) ) ;
#82829=CARTESIAN_POINT ( 'NONE',  ( 37.14004552369136292, -277.4881418609043067, -271.5847058174951485 ) ) ;
#82830=CARTESIAN_POINT ( 'NONE',  ( 5.349099744935768896, -290.7142536620367537, -209.3158710174173223 ) ) ;
#82831=CARTESIAN_POINT ( 'NONE',  ( -94.26682881378687284, -279.7248798894365791, -320.3594700176080892 ) ) ;
#82832=ORIENTED_EDGE ( 'NONE', *, *, #59261, .F. ) ;
#82833=CARTESIAN_POINT ( 'NONE',  ( -13.50395444968439129, -282.0830317907792164, -339.5209057938412229 ) ) ;
#82834=CARTESIAN_POINT ( 'NONE',  ( -72.68594492187368417, -278.5886958296883336, -338.4365937331575083 ) ) ;
#82835=CARTESIAN_POINT ( 'NONE',  ( 36.09360050014341681, -280.6240876018016479, -292.3440534225474039 ) ) ;
#82836=CARTESIAN_POINT ( 'NONE',  ( 200.9738562183072474, 293.9635619827958521, -68.33775802212525718 ) ) ;
#82837=CARTESIAN_POINT ( 'NONE',  ( 37.01383218315248769, -276.7329161312991346, -289.4418681884037028 ) ) ;
#82839=SHAPE_DEFINITION_REPRESENTATION ( #33796, #49383 ) ;
#82840=CARTESIAN_POINT ( 'NONE',  ( -83.17920394262922912, -274.9576867143214258, -209.2898013239136503 ) ) ;
#82841=CARTESIAN_POINT ( 'NONE',  ( -4.771743288812468897, -297.1233781216987495, -337.9199732462171255 ) ) ;
#82842=ORIENTED_EDGE ( 'NONE', *, *, #72401, .F. ) ;
#82846=CARTESIAN_POINT ( 'NONE',  ( -107.2426829067761531, -291.3382042320095593, -292.6214190276682530 ) ) ;
#82847=CARTESIAN_POINT ( 'NONE',  ( 17.60306940398386999, -288.5842140994150782, -217.7967233374841953 ) ) ;
#82848=CARTESIAN_POINT ( 'NONE',  ( -98.20012630852826874, -289.3390732673936441, -310.8826094177516666 ) ) ;
#82849=CARTESIAN_POINT ( 'NONE',  ( -76.07031722933484730, -285.0572425008053301, -203.8195384250526274 ) ) ;
#82851=CARTESIAN_POINT ( 'NONE',  ( -40.28645832146423089, -281.4896529617341798, -344.1023467206119903 ) ) ;
#82852=CARTESIAN_POINT ( 'NONE',  ( 29.91928312765815434, -288.9954272338254100, -238.9473374250240454 ) ) ;
#82853=CARTESIAN_POINT ( 'NONE',  ( -10.74342010822718052, -281.1788777656065577, -339.1410272446179306 ) ) ;
#82854=CARTESIAN_POINT ( 'NONE',  ( -51.94160243309939773, -281.1767062965874402, -198.2806642820031016 ) ) ;
#82855=CARTESIAN_POINT ( 'NONE',  ( 38.05681653991658209, -288.3125280606246861, -255.9429385616485604 ) ) ;
#82856=CARTESIAN_POINT ( 'NONE',  ( -108.9488124987978210, -279.2365199699106029, -255.7927547593441489 ) ) ;
#82857=CARTESIAN_POINT ( 'NONE',  ( -113.4210864942452162, -289.2291710279001222, -279.7403461860976677 ) ) ;
#82858=CARTESIAN_POINT ( 'NONE',  ( -106.8552068454959283, -284.9347005174121250, -303.1030055861094183 ) ) ;
#82859=CARTESIAN_POINT ( 'NONE',  ( 25.49122324765116687, -287.4561764159402060, -225.9362590690421655 ) ) ;
#82860=CARTESIAN_POINT ( 'NONE',  ( -106.9852210808287225, -284.4288143238493376, -292.2421598638657088 ) ) ;
#82863=CARTESIAN_POINT ( 'NONE',  ( -67.85342050438482886, -293.5163700382292973, -200.9975711372078990 ) ) ;
#82864=CARTESIAN_POINT ( 'NONE',  ( 38.11709185191537586, -292.3968304082155214, -283.0605761411659955 ) ) ;
#82865=CARTESIAN_POINT ( 'NONE',  ( 32.28925653025581255, -274.3088159758841584, -247.5056463809646914 ) ) ;
#82866=CARTESIAN_POINT ( 'NONE',  ( -96.43841348009480896, -295.2378757575384611, -319.5841488532150265 ) ) ;
#82867=CARTESIAN_POINT ( 'NONE',  ( -107.2226762753320628, -289.3398327128709866, -246.9654575967048231 ) ) ;
#82868=CARTESIAN_POINT ( 'NONE',  ( -95.58454925547236769, -294.1568676487491416, -316.0310702710178816 ) ) ;
#82869=CARTESIAN_POINT ( 'NONE',  ( -67.98086079002540316, -292.8457912551282902, -203.6511879908065055 ) ) ;
#82871=CARTESIAN_POINT ( 'NONE',  ( 32.76242524983368298, -291.1984148614406536, -243.0981544195494450 ) ) ;
#82872=CARTESIAN_POINT ( 'NONE',  ( 35.79085035455404551, -295.3380261309167167, -253.6722784129947854 ) ) ;
#82873=CARTESIAN_POINT ( 'NONE',  ( 18.01122167145736341, -289.1752535489105753, -318.3897726907940182 ) ) ;
#82874=CARTESIAN_POINT ( 'NONE',  ( -59.16407481432300131, -279.3131125422462446, -342.4873321041928307 ) ) ;
#82875=CARTESIAN_POINT ( 'NONE',  ( -103.2719060889329370, -276.8351851906664933, -309.4679511510514658 ) ) ;
#82876=CARTESIAN_POINT ( 'NONE',  ( -114.0786925784668426, -271.9725663770910273, -264.6255720052324705 ) ) ;
#82877=CARTESIAN_POINT ( 'NONE',  ( -90.48480492610471515, -277.3726647232768983, -218.1620475782953861 ) ) ;
#82878=CARTESIAN_POINT ( 'NONE',  ( -62.16484288454407192, -275.7693996101311313, -342.4602504512316727 ) ) ;
#82879=CARTESIAN_POINT ( 'NONE',  ( -72.37430366501205015, -294.2107920970579471, -334.9816778319416244 ) ) ;
#82881=CARTESIAN_POINT ( 'NONE',  ( -47.30483389811862338, -298.7252911876861958, -197.8298809920019607 ) ) ;
#82883=CARTESIAN_POINT ( 'NONE',  ( -37.52348523585912687, -287.0744941639107424, -345.7288951395824483 ) ) ;
#82884=CARTESIAN_POINT ( 'NONE',  ( -14.06343239113549082, -274.1960378574045194, -201.1720852124626617 ) ) ;
#82885=CARTESIAN_POINT ( 'NONE',  ( 38.10828887158677247, -287.7444005567593308, -285.7331432216089979 ) ) ;
#82886=CARTESIAN_POINT ( 'NONE',  ( -111.7337341645214224, -274.6947677405504464, -259.2417493320547806 ) ) ;
#82887=CARTESIAN_POINT ( 'NONE',  ( -110.6865639051041370, -294.3600576711411918, -285.2762801390736627 ) ) ;
#82888=CARTESIAN_POINT ( 'NONE',  ( -79.08060362343434235, -282.7970449268407265, -334.8748588072818961 ) ) ;
#82890=CARTESIAN_POINT ( 'NONE',  ( -110.4912698441195857, -276.7652465324424611, -253.7470599693036775 ) ) ;
#82891=CARTESIAN_POINT ( 'NONE',  ( -92.84677292810179949, -290.0277077080850177, -222.3369844751966298 ) ) ;
#82895=CARTESIAN_POINT ( 'NONE',  ( -93.14465668288772804, -289.2502622911157459, -220.2317313248454980 ) ) ;
#82896=CARTESIAN_POINT ( 'NONE',  ( 25.86059285657968587, -276.5547126012588137, -232.3653812212576781 ) ) ;
#82897=CARTESIAN_POINT ( 'NONE',  ( 39.12071280703885634, -282.9718067455380037, -269.9154489091039864 ) ) ;
#82898=CARTESIAN_POINT ( 'NONE',  ( -37.23015791734167834, -296.0736571015398226, -195.0051995546122896 ) ) ;
#82899=CARTESIAN_POINT ( 'NONE',  ( -109.4983578076280537, -284.4019186885770409, -281.7496367240956374 ) ) ;
#82900=CARTESIAN_POINT ( 'NONE',  ( -69.76681120801868019, -275.0418136991972347, -204.3006374325418051 ) ) ;
#82901=CARTESIAN_POINT ( 'NONE',  ( 19.97564167922274336, -275.7143841713226493, -224.8732406555960495 ) ) ;
#82903=CARTESIAN_POINT ( 'NONE',  ( -38.67088039133047062, -285.0689823389383264, -345.3493432741486231 ) ) ;
#82905=CARTESIAN_POINT ( 'NONE',  ( -103.4780545064313344, -271.8984004651559871, -238.7350416819934935 ) ) ;
#82907=CARTESIAN_POINT ( 'NONE',  ( 204.5657207964215445, 292.7458577622498979, -53.99999999999736389 ) ) ;
#82908=CARTESIAN_POINT ( 'NONE',  ( 30.90136434622678152, -293.8455866754657109, -306.0246028885624128 ) ) ;
#82909=CARTESIAN_POINT ( 'NONE',  ( -101.8092751909148745, -286.0269856118743519, -307.9879510425555509 ) ) ;
#82911=CARTESIAN_POINT ( 'NONE',  ( -37.30987171927208834, -277.5523547857346784, -190.3611179825600175 ) ) ;
#82912=CARTESIAN_POINT ( 'NONE',  ( -35.72517803117905544, -276.2295613201834499, -347.1957324716757967 ) ) ;
#82913=CARTESIAN_POINT ( 'NONE',  ( -80.10864855193611334, -288.0200071071984667, -333.4917299870747911 ) ) ;
#82914=CARTESIAN_POINT ( 'NONE',  ( -78.75038536192575123, -285.1415307291730414, -331.3203546768234560 ) ) ;
#82915=CARTESIAN_POINT ( 'NONE',  ( -93.48081967303208728, -279.6349510195247490, -318.5936098536361101 ) ) ;
#82916=CARTESIAN_POINT ( 'NONE',  ( -78.22265636648576503, -286.9390093056048840, -205.8060739570703390 ) ) ;
#82917=CARTESIAN_POINT ( 'NONE',  ( 21.22217843365140766, -282.9079775522235991, -223.5073798014388444 ) ) ;
#82918=CARTESIAN_POINT ( 'NONE',  ( -45.64750751806379725, -277.3212055509485481, -346.9649018755663974 ) ) ;
#82919=CARTESIAN_POINT ( 'NONE',  ( -71.57275758701008783, -277.3252158139546282, -339.3338278740602618 ) ) ;
#82920=CARTESIAN_POINT ( 'NONE',  ( -37.85654053871942892, -299.9658069587518980, -195.9228943259563493 ) ) ;
#82922=CARTESIAN_POINT ( 'NONE',  ( -37.37352853689063892, -282.5519495502701943, -195.3611179825600175 ) ) ;
#82923=CARTESIAN_POINT ( 'NONE',  ( -37.57961816093836660, -296.1887933535771822, -194.5966878062021408 ) ) ;
#82925=CARTESIAN_POINT ( 'NONE',  ( -107.8813114569306748, -277.8086458707166457, -289.3914010959801999 ) ) ;
#82926=CARTESIAN_POINT ( 'NONE',  ( 19.72972639834207698, -276.0599043855773971, -219.1866000003836348 ) ) ;
#82927=CARTESIAN_POINT ( 'NONE',  ( 2.980564240251267982, -288.3618441425858236, -208.2959183258687688 ) ) ;
#82929=CARTESIAN_POINT ( 'NONE',  ( -111.9269719779286305, -298.2763813322272313, -254.1834513782348495 ) ) ;
#82930=CARTESIAN_POINT ( 'NONE',  ( -71.88119407151741314, -296.7036348078074184, -338.7353242168666156 ) ) ;
#82931=CARTESIAN_POINT ( 'NONE',  ( -41.72506823871402304, -293.9970988160546881, -195.6051711001187812 ) ) ;
#82932=CARTESIAN_POINT ( 'NONE',  ( -97.05976604789536566, -277.1702440471496516, -225.2423953955258185 ) ) ;
#82933=CARTESIAN_POINT ( 'NONE',  ( -37.02629225820091818, -281.9762850454551426, -195.9217821460108837 ) ) ;
#82934=CARTESIAN_POINT ( 'NONE',  ( -99.63954569464875988, -295.1868963525335516, -229.5211940012381149 ) ) ;
#82935=CARTESIAN_POINT ( 'NONE',  ( -71.16569700766235940, -285.3542770351278364, -338.1567131140929519 ) ) ;
#82936=CARTESIAN_POINT ( 'NONE',  ( 7.125291890327223321, -285.5941405984553398, -212.0139310223021312 ) ) ;
#82937=CARTESIAN_POINT ( 'NONE',  ( -102.1811274640376865, -256.8422514774185288, -326.3129529855307851 ) ) ;
#82939=CARTESIAN_POINT ( 'NONE',  ( 33.05077913577997606, -286.9623839932718283, -250.9449816543256020 ) ) ;
#82941=CARTESIAN_POINT ( 'NONE',  ( -81.37279428861049269, -284.7148439251893137, -333.2170790613274676 ) ) ;
#82942=CARTESIAN_POINT ( 'NONE',  ( -5.302608857870863446, -274.8190544746449859, -204.7303404095251551 ) ) ;
#82943=CARTESIAN_POINT ( 'NONE',  ( 38.39532273392931927, -286.2015967047595382, -258.7883699367978920 ) ) ;
#82944=CARTESIAN_POINT ( 'NONE',  ( -50.49974841359250632, -290.8082246478630850, -194.8074398836162686 ) ) ;
#82945=CARTESIAN_POINT ( 'NONE',  ( 39.29509305955217968, -282.5595336807039075, -275.6327610395879333 ) ) ;
#82946=CARTESIAN_POINT ( 'NONE',  ( -35.37348967407040590, -281.5965192417962726, -194.0668177912773729 ) ) ;
#82947=CARTESIAN_POINT ( 'NONE',  ( 26.26074999568484358, -281.3122758400177190, -226.9036998771602498 ) ) ;
#82948=CARTESIAN_POINT ( 'NONE',  ( -82.13390479932374433, -287.1952119285918457, -326.4764044574609443 ) ) ;
#82949=CARTESIAN_POINT ( 'NONE',  ( 200.5823919207504957, 289.1423781782043534, -97.54666654485188815 ) ) ;
#82951=CARTESIAN_POINT ( 'NONE',  ( 29.68361825208949512, -277.9938789039737799, -303.7591681900066192 ) ) ;
#82952=CARTESIAN_POINT ( 'NONE',  ( 202.6186562182569446, 295.9433822784108656, -54.00000000003930722 ) ) ;
#82953=CARTESIAN_POINT ( 'NONE',  ( 21.83500341415685142, -278.9458730661058325, -224.8434706309899980 ) ) ;
#82954=CARTESIAN_POINT ( 'NONE',  ( -27.85186621224607606, -296.6935120600264213, -345.8054672735639770 ) ) ;
#82955=CARTESIAN_POINT ( 'NONE',  ( -86.56472507778320846, -295.1066510823423528, -324.4072693970779255 ) ) ;
#82956=CARTESIAN_POINT ( 'NONE',  ( -99.97730205154380201, -290.6520775086311232, -225.6810522372269929 ) ) ;
#82959=CARTESIAN_POINT ( 'NONE',  ( -107.2267193329290507, -295.5256344314885268, -239.3323049370431193 ) ) ;
#82960=CARTESIAN_POINT ( 'NONE',  ( 8.460684806095072119, -286.8126780845325356, -328.2280510906520021 ) ) ;
#82961=CARTESIAN_POINT ( 'NONE',  ( 36.85515211788651868, -295.3816246364115159, -267.9752021470371801 ) ) ;
#82963=CARTESIAN_POINT ( 'NONE',  ( -40.00847226590351369, -287.3331214738880135, -196.9163645589655687 ) ) ;
#82965=CARTESIAN_POINT ( 'NONE',  ( 36.05847788520018327, -294.2102941850820912, -247.8837053059766333 ) ) ;
#82966=CARTESIAN_POINT ( 'NONE',  ( -107.4492024774435066, -284.7721154562861443, -290.9709514711556153 ) ) ;
#82967=CARTESIAN_POINT ( 'NONE',  ( -110.4255970676042722, -295.0566925533191238, -293.3561456304659032 ) ) ;
#82968=CARTESIAN_POINT ( 'NONE',  ( -114.2284332157901616, -291.3440045306941784, -271.2371421148016566 ) ) ;
#82969=CARTESIAN_POINT ( 'NONE',  ( -64.37306049884874426, -292.2011410416391755, -198.2714367176935468 ) ) ;
#82970=CARTESIAN_POINT ( 'NONE',  ( -98.84062306416483068, -290.1748068505127094, -309.6915449088135119 ) ) ;
#82973=CARTESIAN_POINT ( 'NONE',  ( -101.2868036239908776, -298.9538471154485251, -229.7245677050963479 ) ) ;
#82974=CARTESIAN_POINT ( 'NONE',  ( -109.7216363701928969, -271.6649544303252810, -245.2781845875908289 ) ) ;
#82975=CARTESIAN_POINT ( 'NONE',  ( -38.90207356077544176, -282.1309129630747634, -343.5923192902827168 ) ) ;
#82978=CARTESIAN_POINT ( 'NONE',  ( 32.49983504887008934, -274.6451257940422011, -237.9590512205796244 ) ) ;
#82980=CARTESIAN_POINT ( 'NONE',  ( -108.6452998610043323, -294.7879861088735538, -289.0256908439316703 ) ) ;
#82981=CARTESIAN_POINT ( 'NONE',  ( -56.90322168860227237, -279.1673876500581173, -342.0260367288996122 ) ) ;
#82982=CARTESIAN_POINT ( 'NONE',  ( -24.35748700101493824, -272.3590913321365292, -197.2177809007490339 ) ) ;
#82983=CARTESIAN_POINT ( 'NONE',  ( -75.42975153439516589, -298.7374008306391033, -207.5612038908421937 ) ) ;
#82984=CARTESIAN_POINT ( 'NONE',  ( -36.49263605649073838, -299.1426998675393065, -197.0518431955534027 ) ) ;
#82986=CARTESIAN_POINT ( 'NONE',  ( -111.8188846858725327, -297.9486585888502077, -286.4728962416030527 ) ) ;
#82987=CARTESIAN_POINT ( 'NONE',  ( -112.6959634789780154, -270.6084402209360746, -267.5297528916812553 ) ) ;
#82988=CARTESIAN_POINT ( 'NONE',  ( 21.41333505682168692, -294.8125336984953151, -313.8552383768067671 ) ) ;
#82989=CARTESIAN_POINT ( 'NONE',  ( 17.18691141796513477, -291.4238177060104817, -220.8697069695756170 ) ) ;
#82991=CARTESIAN_POINT ( 'NONE',  ( 15.97987084479417597, -275.2763064673926010, -214.8963816891093188 ) ) ;
#82992=CARTESIAN_POINT ( 'NONE',  ( -105.4170100565923178, -273.0726969286934036, -243.8635163332248510 ) ) ;
#82993=CARTESIAN_POINT ( 'NONE',  ( 10.46891458260228625, -284.3761273425995455, -328.6742764961313128 ) ) ;
#82994=CARTESIAN_POINT ( 'NONE',  ( -19.05262094601881273, -281.5064867038660736, -344.7044000765649230 ) ) ;
#82996=CARTESIAN_POINT ( 'NONE',  ( -100.5457617325614166, -283.2447090212887701, -307.2101115010094645 ) ) ;
#82997=CARTESIAN_POINT ( 'NONE',  ( -112.5220644747407022, -282.5211962470778531, -272.7645800835308023 ) ) ;
#82998=CARTESIAN_POINT ( 'NONE',  ( -8.524532518911451362, -275.2421546850213758, -338.0869956019382698 ) ) ;
#82999=CARTESIAN_POINT ( 'NONE',  ( 37.14632992430246361, -283.6701436698289172, -279.5379070930167700 ) ) ;
#83002=CARTESIAN_POINT ( 'NONE',  ( -78.39324101171074233, -271.9093927553378762, -206.1644560332355525 ) ) ;
#83003=CARTESIAN_POINT ( 'NONE',  ( -112.5501289269125209, -280.5363918658530338, -271.6041192208650159 ) ) ;
#83005=CARTESIAN_POINT ( 'NONE',  ( -112.0671467456183734, -286.6194417750330103, -258.8161717505068395 ) ) ;
#83006=ORIENTED_EDGE ( 'NONE', *, *, #65700, .F. ) ;
#83008=CARTESIAN_POINT ( 'NONE',  ( -5.899829542312970965, -286.6387064778318177, -338.4661970954428512 ) ) ;
#83010=CARTESIAN_POINT ( 'NONE',  ( -103.1308485592454076, -294.9069897288606512, -303.0170454538719014 ) ) ;
#83011=CARTESIAN_POINT ( 'NONE',  ( -78.88494953664221043, -287.7578247875727584, -331.9455625082819665 ) ) ;
#83012=CARTESIAN_POINT ( 'NONE',  ( 168.1488725781630649, 234.1813984995739588, -193.4213935641190858 ) ) ;
#83013=CARTESIAN_POINT ( 'NONE',  ( -97.21595800675819987, -293.9342288314658731, -315.5494601618863157 ) ) ;
#83014=CARTESIAN_POINT ( 'NONE',  ( -15.59237409132607688, -284.8083609738938549, -197.1647500704050913 ) ) ;
#83015=CARTESIAN_POINT ( 'NONE',  ( -11.48170766011693544, -281.9946934155672125, -201.1861644424373878 ) ) ;
#83016=CARTESIAN_POINT ( 'NONE',  ( -89.75560929285978773, -282.0189167110928565, -325.4492489382009808 ) ) ;
#83017=CARTESIAN_POINT ( 'NONE',  ( -86.72937967292880046, -289.7616654799782054, -324.1870839085988223 ) ) ;
#83018=CARTESIAN_POINT ( 'NONE',  ( -62.52753188734794065, -281.1433267972766430, -201.1621955814928242 ) ) ;
#83019=CARTESIAN_POINT ( 'NONE',  ( -68.60154206500193652, -280.4332986687152243, -204.2141300721354469 ) ) ;
#83020=CARTESIAN_POINT ( 'NONE',  ( 28.92847167474525705, -290.0074261846993409, -306.3405109671757600 ) ) ;
#83021=CARTESIAN_POINT ( 'NONE',  ( -100.7518688048407256, -297.2957874581618967, -226.6555638329493263 ) ) ;
#83023=CARTESIAN_POINT ( 'NONE',  ( -3.826106466615454504, -274.4821253856649719, -201.0234172720022627 ) ) ;
#83024=CARTESIAN_POINT ( 'NONE',  ( -110.9019598376697786, -292.6994204338203076, -257.3873030900396088 ) ) ;
#83026=CARTESIAN_POINT ( 'NONE',  ( 10.59707575819634329, -277.1948066931274184, -210.1954327657594490 ) ) ;
#83028=CARTESIAN_POINT ( 'NONE',  ( -7.330646697743163465, -274.6593686421707616, -339.2906697189735610 ) ) ;
#83030=CARTESIAN_POINT ( 'NONE',  ( -8.707763106063518777, -293.0836862690555336, -341.0324289061744025 ) ) ;
#83031=CARTESIAN_POINT ( 'NONE',  ( 2.993087487901384680, -273.9577666961080809, -209.3334325535352320 ) ) ;
#83032=CARTESIAN_POINT ( 'NONE',  ( -109.8577604937471506, -291.9008344051939048, -283.4809023799742818 ) ) ;
#83033=CARTESIAN_POINT ( 'NONE',  ( 23.42943796244891175, -283.8930458574305362, -312.6085177774449448 ) ) ;
#83035=CARTESIAN_POINT ( 'NONE',  ( -111.9858188822964138, -291.7715394737080032, -286.6970241632299121 ) ) ;
#83036=CARTESIAN_POINT ( 'NONE',  ( -107.9187043993905490, -292.2453704535353722, -240.8283439907328045 ) ) ;
#83037=CARTESIAN_POINT ( 'NONE',  ( 34.32397093922029541, -293.5687509408299434, -284.2546990543729635 ) ) ;
#83038=CARTESIAN_POINT ( 'NONE',  ( 16.44658606462402517, -288.8167080039955863, -218.0942937371492292 ) ) ;
#83039=CARTESIAN_POINT ( 'NONE',  ( 13.68237696362719191, -282.5272890713608263, -328.0996179833335873 ) ) ;
#83040=CARTESIAN_POINT ( 'NONE',  ( -97.08016457353026851, -295.2617128351114388, -224.0733024426773170 ) ) ;
#83041=CARTESIAN_POINT ( 'NONE',  ( 11.49096128488237412, -282.2299005179619371, -329.9647351284985461 ) ) ;
#83042=CARTESIAN_POINT ( 'NONE',  ( 35.72633326637648565, -277.3343530123499932, -255.0374513298922921 ) ) ;
#83043=CARTESIAN_POINT ( 'NONE',  ( -92.05005921254146983, -298.4090924074129703, -314.0302885647153062 ) ) ;
#83045=CARTESIAN_POINT ( 'NONE',  ( -81.84026780938299339, -275.7908411482873134, -331.6814486432688796 ) ) ;
#83047=CARTESIAN_POINT ( 'NONE',  ( -78.41639808493620478, -283.1293856672517109, -330.7834452240858809 ) ) ;
#83048=CARTESIAN_POINT ( 'NONE',  ( -56.47240186498728320, -281.0161232702524217, -196.1307622278391989 ) ) ;
#83049=CARTESIAN_POINT ( 'NONE',  ( 39.34329278359203386, -286.5542387049203512, -265.8442266619545649 ) ) ;
#83050=CARTESIAN_POINT ( 'NONE',  ( -11.93309691514147453, -294.1474676518147362, -200.7911995146945117 ) ) ;
#83051=CARTESIAN_POINT ( 'NONE',  ( 36.85126141049806847, -276.9320584853339824, -252.9307410571222761 ) ) ;
#83052=CARTESIAN_POINT ( 'NONE',  ( 38.82465294507983344, -276.7698049657901720, -262.6135236975884482 ) ) ;
#83053=CARTESIAN_POINT ( 'NONE',  ( -78.63375078936265083, -277.4585620216481630, -330.6220619314908049 ) ) ;
#83054=CARTESIAN_POINT ( 'NONE',  ( -63.74969564120401344, -299.7073753036743256, -200.2873878286791864 ) ) ;
#83055=CARTESIAN_POINT ( 'NONE',  ( -33.11014011545605484, -284.1052760850298000, -195.5964455488650344 ) ) ;
#83056=CARTESIAN_POINT ( 'NONE',  ( -47.73633428001114964, -291.5902842358125326, -194.0335167560572813 ) ) ;
#83057=CARTESIAN_POINT ( 'NONE',  ( -112.3422361346675586, -291.9811542265598518, -283.9017077909066415 ) ) ;
#83058=CARTESIAN_POINT ( 'NONE',  ( 35.02127691032686840, -292.3172283709896533, -258.5426149853789752 ) ) ;
#83060=CARTESIAN_POINT ( 'NONE',  ( 15.04748646970957360, -291.3482983868901783, -214.6649011981226920 ) ) ;
#83061=CARTESIAN_POINT ( 'NONE',  ( 21.01325545229452274, -292.6026496572957285, -226.4659400462186341 ) ) ;
#83063=CARTESIAN_POINT ( 'NONE',  ( -31.83519022091833151, -290.0640028260339705, -346.9064091881161289 ) ) ;
#83064=CARTESIAN_POINT ( 'NONE',  ( -66.11745521326328401, -280.3167409480962533, -203.1473952358238364 ) ) ;
#83065=CARTESIAN_POINT ( 'NONE',  ( -60.04341622400809797, -296.6851199696344565, -197.0519856812748003 ) ) ;
#83066=CARTESIAN_POINT ( 'NONE',  ( -35.15945291713916276, -286.7302549345412217, -193.4808949795269939 ) ) ;
#83067=CARTESIAN_POINT ( 'NONE',  ( -7.355283648241591088, -286.7679202101279543, -199.4062489621444456 ) ) ;
#83068=CARTESIAN_POINT ( 'NONE',  ( -99.62957132219536049, -285.4115477470588189, -232.1556042676293998 ) ) ;
#83069=CARTESIAN_POINT ( 'NONE',  ( 189.4474627607228001, 271.4776447363245779, -139.5738757705058788 ) ) ;
#83070=CARTESIAN_POINT ( 'NONE',  ( -79.02728084768597228, -207.4829129746956653, -355.6029576119787521 ) ) ;
#83071=CARTESIAN_POINT ( 'NONE',  ( -22.36693251778569547, -108.5985266847460622, -358.9081768719106549 ) ) ;
#83072=CARTESIAN_POINT ( 'NONE',  ( -11.20588496726879946, -275.8997874512112958, -338.6950106925331738 ) ) ;
#83073=CARTESIAN_POINT ( 'NONE',  ( -4.941793710671096740, -275.5355755799877784, -336.1357850067452091 ) ) ;
#83074=CARTESIAN_POINT ( 'NONE',  ( -108.8290931161916575, -296.4225312617581949, -241.7736542776215742 ) ) ;
#83075=CARTESIAN_POINT ( 'NONE',  ( -110.3569350145632484, -272.0556378214883466, -283.7581280487278264 ) ) ;
#83077=CARTESIAN_POINT ( 'NONE',  ( -82.27029601463505060, -276.3359953019448199, -332.2862303618889541 ) ) ;
#83078=CARTESIAN_POINT ( 'NONE',  ( -66.22903647347109768, -275.4288700148807720, -202.2179171935093507 ) ) ;
#83079=CARTESIAN_POINT ( 'NONE',  ( -107.4561191903716093, -291.3165651887640593, -249.7750975122339696 ) ) ;
#83080=CARTESIAN_POINT ( 'NONE',  ( -58.79640981861882665, -296.1254943504083599, -344.1990505925075468 ) ) ;
#83081=CARTESIAN_POINT ( 'NONE',  ( -80.59561074974467942, -297.9754200226536227, -206.6682434208644565 ) ) ;
#83082=CARTESIAN_POINT ( 'NONE',  ( 19.69509471483855378, -294.3626145774609313, -315.9420383682352735 ) ) ;
#83084=CARTESIAN_POINT ( 'NONE',  ( -4.596351126262481657, -278.5443058365432307, -338.4712830068449421 ) ) ;
#83086=CARTESIAN_POINT ( 'NONE',  ( 31.96875707627194885, -280.6296010688855631, -236.8381183533995511 ) ) ;
#83087=CARTESIAN_POINT ( 'NONE',  ( 1.004810213960826593, -277.4683479495817551, -332.8142493194610552 ) ) ;
#83088=CARTESIAN_POINT ( 'NONE',  ( -6.959009817387207697, -278.4190625673017507, -340.0233484117898684 ) ) ;
#83089=CARTESIAN_POINT ( 'NONE',  ( 52.59173577772707375, -297.7742714233109496, -196.7942471513891292 ) ) ;
#83091=CARTESIAN_POINT ( 'NONE',  ( -108.8876706831409678, -278.9109054952037923, -255.8009551424368908 ) ) ;
#83092=CARTESIAN_POINT ( 'NONE',  ( 13.84926579877209107, -275.5511103788024343, -212.9869368845743338 ) ) ;
#83093=CARTESIAN_POINT ( 'NONE',  ( -41.74899674898752977, -287.7913852216785813, -346.7540565012317302 ) ) ;
#83094=CARTESIAN_POINT ( 'NONE',  ( 0.1723937790587578844, -276.5517316171739139, -205.4024613651931190 ) ) ;
#83096=CARTESIAN_POINT ( 'NONE',  ( -98.25076229449304321, -289.1876783259443187, -310.9140157406871481 ) ) ;
#83097=CARTESIAN_POINT ( 'NONE',  ( -91.82491323006232165, -284.6481593370122027, -216.0942563031399004 ) ) ;
#83098=CARTESIAN_POINT ( 'NONE',  ( 36.57684789031566197, -279.8407252482076046, -274.1057501538825818 ) ) ;
#83099=CARTESIAN_POINT ( 'NONE',  ( 34.21890914036310249, -280.3521316485039279, -287.5743394025379303 ) ) ;
#83100=CARTESIAN_POINT ( 'NONE',  ( -96.07850890135850364, -283.2641342540224514, -224.6096781897254573 ) ) ;
#83102=CARTESIAN_POINT ( 'NONE',  ( -54.48590238382975315, -291.2724506337452226, -343.4280832037434266 ) ) ;
#83103=CARTESIAN_POINT ( 'NONE',  ( -71.13808908855099844, -280.8007881666577532, -205.1937899692240137 ) ) ;
#83105=CARTESIAN_POINT ( 'NONE',  ( 28.60453745795705416, -279.4503587958092226, -232.1834522322942576 ) ) ;
#83106=CARTESIAN_POINT ( 'NONE',  ( -9.283698933093397443, -294.4191020254279465, -200.8071876931842326 ) ) ;
#83107=CARTESIAN_POINT ( 'NONE',  ( -35.33995882435181102, -278.3167865270415859, -194.3878551397247065 ) ) ;
#83109=CARTESIAN_POINT ( 'NONE',  ( -7.458403146126411976, -277.3010543065921638, -337.0760430741235041 ) ) ;
#83110=CARTESIAN_POINT ( 'NONE',  ( -16.62214569753492910, -284.7853767098214348, -342.6697022834584345 ) ) ;
#83112=CARTESIAN_POINT ( 'NONE',  ( -77.35275394717345421, -291.5040294900244362, -334.5191752487101553 ) ) ;
#83113=CARTESIAN_POINT ( 'NONE',  ( 22.87174090187753706, -286.1090246389712206, -222.6065031546506816 ) ) ;
#83114=CARTESIAN_POINT ( 'NONE',  ( -52.51455800951686825, -290.2545689538642932, -198.0852149254908454 ) ) ;
#83116=CARTESIAN_POINT ( 'NONE',  ( 36.19198120010537423, -274.2533343577543405, -271.6099473374693503 ) ) ;
#83117=CARTESIAN_POINT ( 'NONE',  ( 30.61137758267051723, -292.0871399327428435, -300.2483177050472136 ) ) ;
#83120=CARTESIAN_POINT ( 'NONE',  ( -102.6126562036653525, -289.5537977832203183, -230.7319518079767988 ) ) ;
#83121=CARTESIAN_POINT ( 'NONE',  ( -40.02317025167526765, -287.6180297807639477, -196.6098458938413955 ) ) ;
#83122=CARTESIAN_POINT ( 'NONE',  ( -51.51851457042311466, -287.4709339847963747, -345.0135924471754834 ) ) ;
#83123=CARTESIAN_POINT ( 'NONE',  ( -17.02649037111903141, -287.7447841529243533, -199.5783122343772504 ) ) ;
#83125=CARTESIAN_POINT ( 'NONE',  ( 7.016729896633526309, -287.4763416801692983, -212.1169524188645994 ) ) ;
#83126=CARTESIAN_POINT ( 'NONE',  ( 23.47182552106948350, -294.9283187751506148, -225.8625572963901789 ) ) ;
#83127=CARTESIAN_POINT ( 'NONE',  ( -17.75518393683089613, -274.8813058344071578, -343.3383923823524242 ) ) ;
#83128=CARTESIAN_POINT ( 'NONE',  ( -75.32207260113149516, -277.8775116613626324, -337.3180862408706275 ) ) ;
#83129=CARTESIAN_POINT ( 'NONE',  ( -61.21007982153145122, -289.8246126396358022, -198.6149119826060030 ) ) ;
#83130=CARTESIAN_POINT ( 'NONE',  ( -68.67252482324978757, -279.6516401569736558, -200.0091219581084374 ) ) ;
#83131=CARTESIAN_POINT ( 'NONE',  ( -76.08545204440164866, -299.5120923517177403, -206.4986058663844801 ) ) ;
#83133=CARTESIAN_POINT ( 'NONE',  ( -112.3076814564642376, -282.5809905178211920, -268.1022932347049732 ) ) ;
#83135=CARTESIAN_POINT ( 'NONE',  ( -91.89133863413029246, -275.9799916348003990, -320.7867117569232960 ) ) ;
#83136=CARTESIAN_POINT ( 'NONE',  ( 36.45301858854293187, -279.7248558642858143, -283.8241143756725364 ) ) ;
#83138=CARTESIAN_POINT ( 'NONE',  ( 22.95814458870818342, -274.6623591738508026, -317.1437880219412477 ) ) ;
#83139=CARTESIAN_POINT ( 'NONE',  ( -66.30800298652690117, -296.9585538622890795, -338.1229143897916742 ) ) ;
#83140=CARTESIAN_POINT ( 'NONE',  ( 28.03427491092630675, -280.9995990395029821, -310.5550497094070579 ) ) ;
#83141=CARTESIAN_POINT ( 'NONE',  ( -110.6099278948500881, -297.5147316574928027, -268.7396085574501967 ) ) ;
#83142=CARTESIAN_POINT ( 'NONE',  ( -108.4365821937787047, -298.2297614479181789, -241.9553379311838910 ) ) ;
#83143=CARTESIAN_POINT ( 'NONE',  ( 13.51442350090612265, -274.4552300858728131, -217.9612880576198108 ) ) ;
#83144=CARTESIAN_POINT ( 'NONE',  ( 22.12412568436829119, -296.1785539594726515, -316.0857227883710721 ) ) ;
#83145=CARTESIAN_POINT ( 'NONE',  ( 0.2819371970451695630, -286.7055900410825302, -203.1637669365159411 ) ) ;
#83146=CARTESIAN_POINT ( 'NONE',  ( -7.090014464466213973, -274.7990905942303925, -339.8383779355673937 ) ) ;
#83147=CARTESIAN_POINT ( 'NONE',  ( -43.18441260890356403, -288.9573296845708796, -347.1391273040750889 ) ) ;
#83148=CARTESIAN_POINT ( 'NONE',  ( 33.92730608622555621, -286.8325603911933968, -287.2174877620875577 ) ) ;
#83149=CARTESIAN_POINT ( 'NONE',  ( -110.9568600721551661, -288.7370523765573012, -255.9482898287885746 ) ) ;
#83151=CARTESIAN_POINT ( 'NONE',  ( 180.5468918863934960, 256.3577768311903355, -167.2605672291198857 ) ) ;
#83152=CARTESIAN_POINT ( 'NONE',  ( -74.75279405581906644, -289.0723286309776654, -333.1324787612658156 ) ) ;
#83154=CARTESIAN_POINT ( 'NONE',  ( -105.5695066678691774, -285.0372381067398919, -305.6592552194999257 ) ) ;
#83155=CARTESIAN_POINT ( 'NONE',  ( 26.30455555904806531, -292.0426190136563491, -227.3493617645108600 ) ) ;
#83156=CARTESIAN_POINT ( 'NONE',  ( 5.715257828289471931, -282.2251864295674295, -207.4918982849529527 ) ) ;
#83157=CARTESIAN_POINT ( 'NONE',  ( -33.95397479660803697, -281.4091037548707845, -193.9293079117428817 ) ) ;
#83159=CARTESIAN_POINT ( 'NONE',  ( -36.19566085279808476, -282.8707060976041134, -343.3521215276085172 ) ) ;
#83160=CARTESIAN_POINT ( 'NONE',  ( -9.215319398998989442, -278.6846286859714041, -339.9013645283562823 ) ) ;
#83161=CARTESIAN_POINT ( 'NONE',  ( -75.77990528800914660, -297.5541807025517187, -203.5803301442099382 ) ) ;
#83162=CARTESIAN_POINT ( 'NONE',  ( -2.695874784059958618, -275.8356015078776409, -205.5466885305193898 ) ) ;
#83163=CARTESIAN_POINT ( 'NONE',  ( -33.39685296893049582, -290.1221380521362221, -195.8078522684061227 ) ) ;
#83165=CARTESIAN_POINT ( 'NONE',  ( -40.51765895786904537, -296.9316393825748150, -197.1082309030722968 ) ) ;
#83168=CARTESIAN_POINT ( 'NONE',  ( -97.75757782972854670, -287.0688954467431131, -226.8510209296899234 ) ) ;
#83169=CARTESIAN_POINT ( 'NONE',  ( -34.85085611945666528, -296.1012129746785035, -347.0115465967681985 ) ) ;
#83170=CARTESIAN_POINT ( 'NONE',  ( -99.70059961858143538, -285.7296285267968869, -232.1167816535811141 ) ) ;
#83172=CARTESIAN_POINT ( 'NONE',  ( -54.09162016184902200, -276.3207675419643010, -345.3306141815919545 ) ) ;
#83173=CARTESIAN_POINT ( 'NONE',  ( -74.63673230796331381, -292.2206297008740421, -203.1123755302712368 ) ) ;
#83174=CARTESIAN_POINT ( 'NONE',  ( -54.65890307532110626, -283.9714749688913571, -196.6019154390307619 ) ) ;
#83176=CARTESIAN_POINT ( 'NONE',  ( 21.29158347836460052, -293.2125577443698035, -220.4623054196183034 ) ) ;
#83177=CARTESIAN_POINT ( 'NONE',  ( -92.42488083952731870, -290.2014559514655048, -318.3734115160648912 ) ) ;
#83180=CARTESIAN_POINT ( 'NONE',  ( -69.70536949854505337, -196.1875009344347802, -356.7257175233714861 ) ) ;
#83182=CARTESIAN_POINT ( 'NONE',  ( -112.8047494735694158, -286.2194742402294310, -258.6968085365660954 ) ) ;
#83183=CARTESIAN_POINT ( 'NONE',  ( -114.2704648735229114, -294.0523547857347353, -270.3284710469133074 ) ) ;
#83185=CARTESIAN_POINT ( 'NONE',  ( 18.20771260330259977, -279.7938751577332823, -222.5036913694277700 ) ) ;
#83186=CARTESIAN_POINT ( 'NONE',  ( 8.225130196732044041, -276.1147838858450427, -332.4707111938078015 ) ) ;
#83187=CARTESIAN_POINT ( 'NONE',  ( -19.11200047120404122, -282.2873267007680624, -197.7285527077597180 ) ) ;
#83188=CARTESIAN_POINT ( 'NONE',  ( -97.05825111094482338, -248.4111539963268740, -332.8678862503371079 ) ) ;
#83189=CARTESIAN_POINT ( 'NONE',  ( -90.04496921573739598, -282.3537317053323932, -325.7597341201185372 ) ) ;
#83190=CARTESIAN_POINT ( 'NONE',  ( -75.54064640864875457, -283.5599502960607197, -206.2308809204665181 ) ) ;
#83191=CARTESIAN_POINT ( 'NONE',  ( -113.1065001290297545, -274.4122686959622115, -270.3847523717674335 ) ) ;
#83192=CARTESIAN_POINT ( 'NONE',  ( -107.6603347381303024, -296.7825687261477583, -290.1923576904333686 ) ) ;
#83194=CARTESIAN_POINT ( 'NONE',  ( -12.07503723466268397, -291.0726482404612057, -201.2935448514444943 ) ) ;
#83195=CARTESIAN_POINT ( 'NONE',  ( 20.74870263431859740, -276.8855229691156410, -320.7677336948189009 ) ) ;
#83196=CARTESIAN_POINT ( 'NONE',  ( 18.99885335402941422, -274.8942946963477425, -223.9419190091889504 ) ) ;
#83197=CARTESIAN_POINT ( 'NONE',  ( 32.27824904882037771, -274.0578960981491150, -238.0701051869069431 ) ) ;
#83199=CARTESIAN_POINT ( 'NONE',  ( -19.80690828132705050, -272.2772748964343350, -197.3868958706597141 ) ) ;
#83201=CARTESIAN_POINT ( 'NONE',  ( 27.61467143157695148, -295.5088486365418134, -310.7007898283400777 ) ) ;
#83204=CARTESIAN_POINT ( 'NONE',  ( -7.113509023457820213, -283.7256787409455683, -337.1617350806279205 ) ) ;
#83205=CARTESIAN_POINT ( 'NONE',  ( 32.23597609400210473, -282.9175547939278772, -239.8173627624601636 ) ) ;
#83206=CARTESIAN_POINT ( 'NONE',  ( -95.03239482664280047, -284.5326697714195916, -225.4445098187927385 ) ) ;
#83207=CARTESIAN_POINT ( 'NONE',  ( -10.98718220638100362, -275.1026202818105730, -339.2949978994091111 ) ) ;
#83208=CARTESIAN_POINT ( 'NONE',  ( -10.50753251409707012, -284.5588702689336174, -339.6311675518573452 ) ) ;
#83209=CARTESIAN_POINT ( 'NONE',  ( -94.15278944238026781, -276.3727118290278781, -317.3192374782005345 ) ) ;
#83210=CARTESIAN_POINT ( 'NONE',  ( 9.672831515439035854, -275.7963067823124561, -214.0464532056879534 ) ) ;
#83212=CARTESIAN_POINT ( 'NONE',  ( -77.41704251632816636, -280.3322169371054997, -204.7394245984010865 ) ) ;
#83217=CARTESIAN_POINT ( 'NONE',  ( -105.5771099020245316, -286.8419108962791029, -237.4334042637140669 ) ) ;
#83218=CARTESIAN_POINT ( 'NONE',  ( -41.05762463071861390, -294.2972409424061766, -343.4407619019840467 ) ) ;
#83219=CARTESIAN_POINT ( 'NONE',  ( -87.32448557239666798, -289.0761422646986603, -328.8693568803246876 ) ) ;
#83220=CARTESIAN_POINT ( 'NONE',  ( 32.34607846310996848, -286.1194317034921824, -295.2927751172559283 ) ) ;
#83221=CARTESIAN_POINT ( 'NONE',  ( -39.97698862683193255, -284.5931181933934795, -196.8190880071194329 ) ) ;
#83222=CARTESIAN_POINT ( 'NONE',  ( -110.7979327074476998, -288.6740734437386209, -279.4251076248659729 ) ) ;
#83223=CARTESIAN_POINT ( 'NONE',  ( -107.7401714905424228, -286.0325956486889822, -249.4197057840079026 ) ) ;
#83224=CARTESIAN_POINT ( 'NONE',  ( -15.20496157192699904, -274.7654898958717808, -342.0741607336552192 ) ) ;
#83225=CARTESIAN_POINT ( 'NONE',  ( 34.11121775428021152, -285.6138032643681868, -243.8862064574834676 ) ) ;
#83226=CARTESIAN_POINT ( 'NONE',  ( -104.7278169973263573, -298.9863765777511162, -237.4352634164672509 ) ) ;
#83227=CARTESIAN_POINT ( 'NONE',  ( 35.36446571222547419, -285.7965889165869839, -289.4357576458212407 ) ) ;
#83228=CARTESIAN_POINT ( 'NONE',  ( 32.19624995882173835, -282.1874816862875832, -247.2256841327707093 ) ) ;
#83229=CARTESIAN_POINT ( 'NONE',  ( -97.54510290562218700, -291.9386487239567600, -315.3888236536990348 ) ) ;
#83232=CARTESIAN_POINT ( 'NONE',  ( -105.8502771178793296, -298.0565854005219535, -302.2341328069030055 ) ) ;
#83233=CARTESIAN_POINT ( 'NONE',  ( -86.78404811331400026, -277.3642737483932592, -213.9655962481994322 ) ) ;
#83234=CARTESIAN_POINT ( 'NONE',  ( -58.88359884752441076, -290.9775192637200121, -196.6040476799545900 ) ) ;
#83235=CARTESIAN_POINT ( 'NONE',  ( -108.7487592832080168, -294.7079926242935244, -289.0517460242874677 ) ) ;
#83236=CARTESIAN_POINT ( 'NONE',  ( 19.72443105625738013, -280.8880721409860257, -316.6918569046043785 ) ) ;
#83237=CARTESIAN_POINT ( 'NONE',  ( -2.212929956298244960, -272.6007963000595282, -204.7312184997753661 ) ) ;
#83238=CARTESIAN_POINT ( 'NONE',  ( 20.92435662976772548, -295.4936783009602550, -315.1735815786920512 ) ) ;
#83239=CARTESIAN_POINT ( 'NONE',  ( -54.49178911615188525, -300.3376638359845288, -195.3683826091709363 ) ) ;
#83240=CARTESIAN_POINT ( 'NONE',  ( 52.59015588275923392, -297.6385992399109455, -194.0771794660524279 ) ) ;
#83241=CARTESIAN_POINT ( 'NONE',  ( -27.89631698261259629, -293.1737967659688024, -345.8110473453802456 ) ) ;
#83242=CARTESIAN_POINT ( 'NONE',  ( 2.544748863795425198, -294.0233065930323164, -208.4586566532220218 ) ) ;
#83244=CARTESIAN_POINT ( 'NONE',  ( 33.46190228742342043, -294.1122826943876021, -251.9369053158165741 ) ) ;
#83245=AXIS2_PLACEMENT_3D ( 'NONE', #89210, #31940, #60829 ) ;
#83247=CARTESIAN_POINT ( 'NONE',  ( -87.25143057011788983, -281.7633821609863389, -326.8881012458639930 ) ) ;
#83248=CARTESIAN_POINT ( 'NONE',  ( -75.65805633681154063, -295.5786477249818631, -332.5558444531047826 ) ) ;
#83249=CARTESIAN_POINT ( 'NONE',  ( 38.14554913369389766, -281.7420990074488145, -285.5491132054527270 ) ) ;
#83251=CARTESIAN_POINT ( 'NONE',  ( -58.48501760427461704, -282.9848260694627697, -344.4348728664098758 ) ) ;
#83252=CARTESIAN_POINT ( 'NONE',  ( -99.65095508441373795, -287.9905435756493830, -311.8282169226496308 ) ) ;
#83254=CARTESIAN_POINT ( 'NONE',  ( 4.152293452008417596, -280.9841419206805995, -334.4622683585670302 ) ) ;
#83255=CARTESIAN_POINT ( 'NONE',  ( -20.57742128474241738, -287.7622242428591903, -345.2517276494198768 ) ) ;
#83257=CARTESIAN_POINT ( 'NONE',  ( -71.28076103321581058, -297.1081090744941662, -335.9083033716763111 ) ) ;
#83258=CARTESIAN_POINT ( 'NONE',  ( 30.03216182896389341, -277.4481546943553667, -306.5196481849504266 ) ) ;
#83259=CARTESIAN_POINT ( 'NONE',  ( -106.4633666503563347, -278.5335082491939147, -246.6626598034360143 ) ) ;
#83260=CARTESIAN_POINT ( 'NONE',  ( 37.42143541267572715, -293.4883400369601532, -251.9363094721450125 ) ) ;
#83261=CARTESIAN_POINT ( 'NONE',  ( -24.79718615571157514, -280.9733054289794723, -344.9256234413394964 ) ) ;
#83262=CARTESIAN_POINT ( 'NONE',  ( -4.717527877856648288, -291.5514842592104969, -204.7798398768614163 ) ) ;
#83263=CARTESIAN_POINT ( 'NONE',  ( -110.6402949683239285, -294.7566692966816504, -254.4167933054898185 ) ) ;
#83266=CARTESIAN_POINT ( 'NONE',  ( -7.969317369887636282, -294.1643260986725181, -337.2720272974965496 ) ) ;
#83268=CARTESIAN_POINT ( 'NONE',  ( -102.0172624299487154, -294.4809262143061801, -239.1787733560258289 ) ) ;
#83269=CARTESIAN_POINT ( 'NONE',  ( -114.1798439490726054, -271.7853104079259765, -267.4894666277526198 ) ) ;
#83270=CARTESIAN_POINT ( 'NONE',  ( 37.57702599966744827, -279.5438913507804841, -258.7290094800859492 ) ) ;
#83271=CARTESIAN_POINT ( 'NONE',  ( -36.58722580065883534, -287.3766033886709010, -193.8450319251169276 ) ) ;
#83272=CARTESIAN_POINT ( 'NONE',  ( -29.17522936735944938, -288.7790977884083077, -342.9028904988959425 ) ) ;
#83273=CARTESIAN_POINT ( 'NONE',  ( -106.9124004078946939, -279.7502123630232518, -294.8185464424838074 ) ) ;
#83274=CARTESIAN_POINT ( 'NONE',  ( -110.9886143634434887, -274.2238866686519714, -264.8740468337414882 ) ) ;
#83275=CARTESIAN_POINT ( 'NONE',  ( -108.3528706729627515, -277.5914034571713387, -251.7498901552513928 ) ) ;
#83277=CARTESIAN_POINT ( 'NONE',  ( -114.3417001280813849, -272.3854989540131442, -270.3590004217965088 ) ) ;
#83278=CARTESIAN_POINT ( 'NONE',  ( -107.3793003533697146, -292.1429072489794976, -295.5811249467953985 ) ) ;
#83279=CARTESIAN_POINT ( 'NONE',  ( 35.60979886873431610, -295.4335015497329664, -292.5518220834818521 ) ) ;
#83281=CARTESIAN_POINT ( 'NONE',  ( -73.58830703904730797, -290.1982105326773080, -333.8584295832638418 ) ) ;
#83284=CARTESIAN_POINT ( 'NONE',  ( 27.01586018128563538, -291.1591126990565499, -230.2818182179555322 ) ) ;
#83285=CARTESIAN_POINT ( 'NONE',  ( -29.06671523562641468, -298.4863826236468185, -193.3818080976452904 ) ) ;
#83288=CARTESIAN_POINT ( 'NONE',  ( -109.2059864757586212, -291.7437069328147459, -296.1736896283744613 ) ) ;
#83289=CARTESIAN_POINT ( 'NONE',  ( 44.71564893372296723, -296.0519495502701943, -270.3284710469131937 ) ) ;
#83290=CARTESIAN_POINT ( 'NONE',  ( -57.92244669427246606, -287.7860059568863562, -198.3595484264738502 ) ) ;
#83291=CARTESIAN_POINT ( 'NONE',  ( -67.78046913888434233, -271.6516253564632279, -201.9840105527592868 ) ) ;
#83292=CARTESIAN_POINT ( 'NONE',  ( -101.9800678583620339, -274.9696152174484496, -233.3359258882194638 ) ) ;
#83293=CARTESIAN_POINT ( 'NONE',  ( 22.98579280248460321, -291.0334856379262760, -226.7285651111565414 ) ) ;
#83294=CARTESIAN_POINT ( 'NONE',  ( -72.25014979657481717, -279.3693141221907013, -337.6192128514094861 ) ) ;
#83296=CARTESIAN_POINT ( 'NONE',  ( 28.23885174087255123, -281.3391539641907002, -302.7727779485226733 ) ) ;
#83297=CARTESIAN_POINT ( 'NONE',  ( 37.60653784183389803, -276.8367109855100239, -286.6784192960640212 ) ) ;
#83298=CARTESIAN_POINT ( 'NONE',  ( 18.87922307554504187, -279.6346889309546100, -218.3301991669989945 ) ) ;
#83299=CARTESIAN_POINT ( 'NONE',  ( 200.9738707121548487, 293.6302286493877318, -68.30388873731220656 ) ) ;
#83300=CARTESIAN_POINT ( 'NONE',  ( 22.56717584958217770, -275.8482591014254695, -222.3429151664357448 ) ) ;
#83303=CARTESIAN_POINT ( 'NONE',  ( -35.55956057785753899, -275.5942169536958204, -194.0622504129907497 ) ) ;
#83304=CARTESIAN_POINT ( 'NONE',  ( -105.5937364680635966, -281.2662352645559167, -254.8156830097664738 ) ) ;
#83306=DIRECTION ( 'NONE',  ( 0.000000000000000000, 0.000000000000000000, -1.000000000000000000 ) ) ;
#83308=CARTESIAN_POINT ( 'NONE',  ( -68.87854996587870460, -290.5565500625998538, -336.5400661233987307 ) ) ;
#83309=CARTESIAN_POINT ( 'NONE',  ( 11.41004590248148531, -288.4771033813177041, -212.0066164215762967 ) ) ;
#83310=CARTESIAN_POINT ( 'NONE',  ( -75.92957757043760125, -288.9310697877745611, -332.4487043634551355 ) ) ;
#83311=CARTESIAN_POINT ( 'NONE',  ( 22.94758027405440615, -286.4194597403190983, -222.5412719806427901 ) ) ;
#83313=CARTESIAN_POINT ( 'NONE',  ( -5.708323508255333856, -281.0290212011087192, -337.0516244364250724 ) ) ;
#83314=CARTESIAN_POINT ( 'NONE',  ( -23.53255292911645924, -290.7343436940137167, -343.3532103296899436 ) ) ;
#83315=CARTESIAN_POINT ( 'NONE',  ( 8.207455521533429277, -280.8963281503307599, -328.3571158065620921 ) ) ;
#83316=CARTESIAN_POINT ( 'NONE',  ( -108.4539811086181373, -280.1112457013910557, -251.7566695546871642 ) ) ;
#83317=CARTESIAN_POINT ( 'NONE',  ( -29.70075918095427170, -277.4452896280946561, -343.0729538277769279 ) ) ;
#83318=CARTESIAN_POINT ( 'NONE',  ( -113.7905917931544195, -289.4081175454489312, -265.5056385191937807 ) ) ;
#83319=CARTESIAN_POINT ( 'NONE',  ( -52.15219579729848220, -286.6701553414141586, -194.9091745017959170 ) ) ;
#83320=CARTESIAN_POINT ( 'NONE',  ( 23.80870509021086789, -287.4212274303690720, -223.6473909717856827 ) ) ;
#83321=CARTESIAN_POINT ( 'NONE',  ( -110.0955936040637795, -284.6398252064130929, -276.3503573813566732 ) ) ;
#83324=CARTESIAN_POINT ( 'NONE',  ( -98.02535698662634900, -291.7989267795626347, -315.7455363306515324 ) ) ;
#83325=CARTESIAN_POINT ( 'NONE',  ( -6.015041406537023683, -293.3337742651395388, -340.1603925314517483 ) ) ;
#83326=CARTESIAN_POINT ( 'NONE',  ( 21.67789180088654177, -274.0053569293037299, -227.0010416776049169 ) ) ;
#83327=CARTESIAN_POINT ( 'NONE',  ( -111.8719108426423929, -295.6628836716047317, -289.3499932580477321 ) ) ;
#83328=CARTESIAN_POINT ( 'NONE',  ( -52.49359440065099136, -290.3345624990209899, -198.1898818989702988 ) ) ;
#83329=CARTESIAN_POINT ( 'NONE',  ( 4.369234031972163201, -292.7208328059975884, -331.5017099258112694 ) ) ;
#83330=CARTESIAN_POINT ( 'NONE',  ( -108.7330864522271128, -291.5336243651678387, -287.4022583451558148 ) ) ;
#83332=CARTESIAN_POINT ( 'NONE',  ( 36.27177948952483177, -291.3564332626361306, -255.0964826588745780 ) ) ;
#83333=CARTESIAN_POINT ( 'NONE',  ( 19.31339685859821742, -296.2347575297886806, -319.5823197403796030 ) ) ;
#83334=CARTESIAN_POINT ( 'NONE',  ( 32.89222662944607833, -288.2191763907642326, -249.5659052442754842 ) ) ;
#83335=CARTESIAN_POINT ( 'NONE',  ( 36.02755172885924395, -277.3117607985875566, -253.1190377707951313 ) ) ;
#83336=CARTESIAN_POINT ( 'NONE',  ( -17.47573911354671594, -275.5962690678069862, -344.3432260255914343 ) ) ;
#83337=CARTESIAN_POINT ( 'NONE',  ( -113.7604456051334409, -272.0080941347234216, -261.7885964075962306 ) ) ;
#83338=CARTESIAN_POINT ( 'NONE',  ( 35.15263811323885079, -273.9861073113754628, -285.2790581522954199 ) ) ;
#83339=CARTESIAN_POINT ( 'NONE',  ( -13.83134329412208174, -278.4393196359653189, -199.6767566697508300 ) ) ;
#83340=CARTESIAN_POINT ( 'NONE',  ( 35.10159219554091692, -276.9160080622418150, -282.4626632348733324 ) ) ;
#83341=CARTESIAN_POINT ( 'NONE',  ( -84.38862496545182523, -276.0868920106904625, -330.3700439172448000 ) ) ;
#83343=CARTESIAN_POINT ( 'NONE',  ( -90.27613212494456718, -273.9297675972762818, -219.9261520788251119 ) ) ;
#83345=CARTESIAN_POINT ( 'NONE',  ( -38.91173403247118756, -287.0918713555852264, -345.6999645357195732 ) ) ;
#83346=CARTESIAN_POINT ( 'NONE',  ( 19.85682786961195845, -274.7450286067314096, -224.9833335238277812 ) ) ;
#83347=CARTESIAN_POINT ( 'NONE',  ( 31.68742154508574771, -287.9919321177838469, -304.5985248271242085 ) ) ;
#83348=CARTESIAN_POINT ( 'NONE',  ( -89.48027949774179035, -289.4299499131792572, -326.9942605120532448 ) ) ;
#83349=CARTESIAN_POINT ( 'NONE',  ( -95.53336798483998393, -275.2068316506991437, -222.7620568408226518 ) ) ;
#83350=CARTESIAN_POINT ( 'NONE',  ( -109.3742783101513538, -294.2904637175404332, -290.6425407325457968 ) ) ;
#83351=CARTESIAN_POINT ( 'NONE',  ( 37.70560280667164932, -280.9568022370764311, -286.9161211083728062 ) ) ;
#83353=CARTESIAN_POINT ( 'NONE',  ( -34.74687298594315621, -278.0844949551296281, -195.3558671629433263 ) ) ;
#83355=CARTESIAN_POINT ( 'NONE',  ( -110.0182797356726212, -289.2112867694162333, -280.7103298263742204 ) ) ;
#83357=CARTESIAN_POINT ( 'NONE',  ( -64.78022087047456523, -289.6937010153351366, -200.5465843163862871 ) ) ;
#83358=CARTESIAN_POINT ( 'NONE',  ( -11.26280442437097129, -275.9182305945000735, -201.3819758647652520 ) ) ;
#83359=CARTESIAN_POINT ( 'NONE',  ( 38.82291841351219119, -282.9001875325752167, -264.2327271565270053 ) ) ;
#83360=CARTESIAN_POINT ( 'NONE',  ( -96.66698164563842965, -271.2698571632007543, -223.5655500793722581 ) ) ;
#83361=CARTESIAN_POINT ( 'NONE',  ( -97.53234923149224755, -283.9761248469291672, -311.7540092301907180 ) ) ;
#83362=CARTESIAN_POINT ( 'NONE',  ( 11.92766407886652047, -276.1778221786436234, -215.6307909317528697 ) ) ;
#83363=CARTESIAN_POINT ( 'NONE',  ( 25.40907944586396638, -275.8375387543028978, -232.6473063329487445 ) ) ;
#83364=CARTESIAN_POINT ( 'NONE',  ( -12.71657381548230248, -286.8144823243158612, -341.8506441788350116 ) ) ;
#83366=CARTESIAN_POINT ( 'NONE',  ( -5.002524092355371543, -284.6265849750445796, -338.0448600208533776 ) ) ;
#83367=CARTESIAN_POINT ( 'NONE',  ( -96.52280491215569214, -272.0767862475556740, -227.0122298766106894 ) ) ;
#83370=CARTESIAN_POINT ( 'NONE',  ( 37.45949928069436652, -293.6146311769580848, -288.6859448864928481 ) ) ;
#83372=CARTESIAN_POINT ( 'NONE',  ( -104.9864642901697067, -286.9502375379933596, -238.6785144397962881 ) ) ;
#83374=CARTESIAN_POINT ( 'NONE',  ( 25.22466315766302358, -272.4094976428775681, -220.5068182859052968 ) ) ;
#83375=CARTESIAN_POINT ( 'NONE',  ( -25.80432594554962122, -276.1059232435649733, -346.3285308453869220 ) ) ;
#83376=CARTESIAN_POINT ( 'NONE',  ( -104.4610361619844952, -288.4807273590805039, -306.4365271129806274 ) ) ;
#83378=CARTESIAN_POINT ( 'NONE',  ( -92.16804384127794947, -285.3739220903968885, -319.6221531244599987 ) ) ;
#83379=CARTESIAN_POINT ( 'NONE',  ( -102.7420114453258719, -279.8467207816627820, -305.0132938261650111 ) ) ;
#83380=CARTESIAN_POINT ( 'NONE',  ( -97.13078241085194975, -286.6193135897519824, -222.7809547257787699 ) ) ;
#83381=CARTESIAN_POINT ( 'NONE',  ( 6.060370705028900851, -282.6412053463523648, -209.1952705386757998 ) ) ;
#83382=CARTESIAN_POINT ( 'NONE',  ( 37.94494193586086794, -275.5160354403257656, -254.1457279098691799 ) ) ;
#83383=CARTESIAN_POINT ( 'NONE',  ( -22.94098218348056051, -276.7062569876982252, -346.0566890567357063 ) ) ;
#83384=CARTESIAN_POINT ( 'NONE',  ( -8.653767693668044103, -296.5939800589054016, -339.0649990813101908 ) ) ;
#83386=CARTESIAN_POINT ( 'NONE',  ( -59.75963548836536887, -295.9045011513117629, -197.9342491449833688 ) ) ;
#83387=CARTESIAN_POINT ( 'NONE',  ( -107.1773006107004136, -277.7736299852884940, -292.0009603506158555 ) ) ;
#83388=CARTESIAN_POINT ( 'NONE',  ( -68.06630080114807413, -298.7378992605416670, -200.0372572020415873 ) ) ;
#83389=CARTESIAN_POINT ( 'NONE',  ( -40.03290297085443683, -287.7780167539228273, -196.3967249096531020 ) ) ;
#83390=CARTESIAN_POINT ( 'NONE',  ( -65.33100169161924953, -296.9315359302708544, -341.3632849548062609 ) ) ;
#83391=CARTESIAN_POINT ( 'NONE',  ( -24.95680792198181308, -296.1027679658405987, -346.0100330594558500 ) ) ;
#83392=CARTESIAN_POINT ( 'NONE',  ( -112.1699763204347704, -292.5411176606045842, -271.2314658782549941 ) ) ;
#83393=CARTESIAN_POINT ( 'NONE',  ( -84.57567925999404679, -277.4001464939907464, -212.2511554480599330 ) ) ;
#83394=CARTESIAN_POINT ( 'NONE',  ( -103.4456679872251925, -280.9300996767619267, -236.0205183911125744 ) ) ;
#83395=CARTESIAN_POINT ( 'NONE',  ( 10.10186817582977348, -296.7303688635369667, -195.9367804121130234 ) ) ;
#83396=CARTESIAN_POINT ( 'NONE',  ( -95.30971361379631901, -285.7446955368546355, -319.1665798725999252 ) ) ;
#83397=CARTESIAN_POINT ( 'NONE',  ( 35.93834548644947802, -286.5174891728832449, -273.7879314718856563 ) ) ;
#83398=CARTESIAN_POINT ( 'NONE',  ( 46.71364630202708668, 11.49618872572055928, -331.6741688793942444 ) ) ;
#83400=CARTESIAN_POINT ( 'NONE',  ( -35.92880368154460058, -285.7370759576803039, -197.3536443206606066 ) ) ;
#83401=ORIENTED_EDGE ( 'NONE', *, *, #78083, .F. ) ;
#83402=CARTESIAN_POINT ( 'NONE',  ( -21.77524475299092899, -283.9367973685962738, -345.4555783370901736 ) ) ;
#83403=CARTESIAN_POINT ( 'NONE',  ( -34.04397020031636600, -274.4280528451893701, -197.4144767702829313 ) ) ;
#83404=CARTESIAN_POINT ( 'NONE',  ( 22.69033527415341922, -285.7068466318258970, -222.7569785289044262 ) ) ;
#83405=CARTESIAN_POINT ( 'NONE',  ( -3.771362608470006705, -281.4255067774773238, -201.3114902957267986 ) ) ;
#83406=CARTESIAN_POINT ( 'NONE',  ( -92.58529693527088966, -280.7991213201947858, -217.6467106564701055 ) ) ;
#83407=CARTESIAN_POINT ( 'NONE',  ( 39.16126474362443588, -281.7726827342077627, -261.3482260640716959 ) ) ;
#83408=CARTESIAN_POINT ( 'NONE',  ( 34.45848030099739390, -291.0523547857347353, -270.3937649182068412 ) ) ;
#83409=CARTESIAN_POINT ( 'NONE',  ( -94.77334838489042568, -240.6273343624868062, -341.9136549172818036 ) ) ;
#83411=CARTESIAN_POINT ( 'NONE',  ( -62.67366924264906913, -275.7218535603614100, -199.9457804022509038 ) ) ;
#83412=CARTESIAN_POINT ( 'NONE',  ( 102.5922281513134919, 116.6502060167416630, -282.7433585466509953 ) ) ;
#83413=CARTESIAN_POINT ( 'NONE',  ( 32.89385920118760964, -279.9032344003597927, -295.7885500806293066 ) ) ;
#83414=CARTESIAN_POINT ( 'NONE',  ( -14.19672073583915406, -294.1082850755699951, -197.9298951725927793 ) ) ;
#83415=CARTESIAN_POINT ( 'NONE',  ( -68.56840588567902728, -294.8222150961618695, -336.4716579983996780 ) ) ;
#83416=CARTESIAN_POINT ( 'NONE',  ( -103.1599465381613072, -290.5814069812535649, -230.4151532101164719 ) ) ;
#83418=CARTESIAN_POINT ( 'NONE',  ( -111.4020735775331445, -294.8891497395210308, -289.2200370318740283 ) ) ;
#83419=CARTESIAN_POINT ( 'NONE',  ( 4.046591436637537065, -286.8845311378838119, -331.5246905276018765 ) ) ;
#83420=CARTESIAN_POINT ( 'NONE',  ( 36.12684947545425018, -295.2745311739885210, -259.7197975918480211 ) ) ;
#83421=CARTESIAN_POINT ( 'NONE',  ( -108.9016642274088582, -285.6472534599096207, -287.1616447437694433 ) ) ;
#83423=CARTESIAN_POINT ( 'NONE',  ( -11.24455104975812425, -293.3251819477607114, -198.1127417469649856 ) ) ;
#83424=CARTESIAN_POINT ( 'NONE',  ( -4.794121284811317274, -283.1037881810158297, -335.7724591498637210 ) ) ;
#83425=CARTESIAN_POINT ( 'NONE',  ( -44.77246218567561442, -293.9390128652876228, -346.6559213921134415 ) ) ;
#83426=CARTESIAN_POINT ( 'NONE',  ( -87.27172989295904415, -290.5301540142922931, -328.8360552638200147 ) ) ;
#83428=CARTESIAN_POINT ( 'NONE',  ( -113.1125059952144767, -291.2116328229413398, -257.0077707773682505 ) ) ;
#83429=CARTESIAN_POINT ( 'NONE',  ( -109.1785398885511995, -290.5476111811140072, -283.3406579493222353 ) ) ;
#83431=CARTESIAN_POINT ( 'NONE',  ( -106.0363124427144754, -297.9968568859628704, -302.3197743487646676 ) ) ;
#83432=CARTESIAN_POINT ( 'NONE',  ( -112.0526032524244897, -271.5597887483050386, -253.4410212040034196 ) ) ;
#83434=CARTESIAN_POINT ( 'NONE',  ( -59.79440787993041084, -278.8128975124869271, -200.5990769741631539 ) ) ;
#83437=CARTESIAN_POINT ( 'NONE',  ( -13.07594815375333930, -273.8668476596614028, -197.3494738136759850 ) ) ;
#83438=CARTESIAN_POINT ( 'NONE',  ( -88.59417177527213028, -295.7975433669884637, -217.3381036303860583 ) ) ;
#83439=CARTESIAN_POINT ( 'NONE',  ( 19.26541006732544759, -278.0840356577512580, -318.3871583984513904 ) ) ;
#83440=CARTESIAN_POINT ( 'NONE',  ( 36.24804142996119083, -273.5650185599660063, -260.5930364160385011 ) ) ;
#83442=CARTESIAN_POINT ( 'NONE',  ( -67.44410390668862476, -296.6610922589126744, -337.3149881339224407 ) ) ;
#83443=CARTESIAN_POINT ( 'NONE',  ( -68.19008139768868659, -298.7169311966987948, -203.8447372838440685 ) ) ;
#83444=DIRECTION ( 'NONE',  ( 1.000000000000000000, 0.000000000000000000, 0.000000000000000000 ) ) ;
#83445=CARTESIAN_POINT ( 'NONE',  ( -110.0304720195537982, -297.8614440644573165, -293.2691992942622505 ) ) ;
#83446=CARTESIAN_POINT ( 'NONE',  ( -112.2252945396787993, -270.6798292912490638, -261.9436308493769729 ) ) ;
#83447=CARTESIAN_POINT ( 'NONE',  ( 35.72294778351895417, -294.1728165033564437, -268.0266173076009295 ) ) ;
#83448=CARTESIAN_POINT ( 'NONE',  ( -107.1243316290799754, -289.4346670870831986, -246.9996270687985316 ) ) ;
#83450=CARTESIAN_POINT ( 'NONE',  ( 38.67594812071207855, -276.1972263816411441, -282.5634380782915400 ) ) ;
#83451=CARTESIAN_POINT ( 'NONE',  ( -34.48315416847574966, -298.4221895734845589, -197.3398065820845773 ) ) ;
#83453=CARTESIAN_POINT ( 'NONE',  ( -19.28750040698190205, -284.8010226849348783, -343.5753643798592520 ) ) ;
#83454=CARTESIAN_POINT ( 'NONE',  ( 8.897359168909336091, -281.1174375276990531, -331.3139494736201982 ) ) ;
#83455=CARTESIAN_POINT ( 'NONE',  ( -77.76838110910631485, -276.9281774339719391, -335.8370374268101273 ) ) ;
#83457=CARTESIAN_POINT ( 'NONE',  ( -90.86655409766818536, -283.0336673584465643, -320.2378834610705667 ) ) ;
#83458=CARTESIAN_POINT ( 'NONE',  ( 36.06937697272130094, -279.7596681679433459, -286.5710787778032795 ) ) ;
#83459=CARTESIAN_POINT ( 'NONE',  ( 22.93814492978057018, -274.7118847282850425, -312.6589417394282577 ) ) ;
#83460=CARTESIAN_POINT ( 'NONE',  ( -71.06402104504375927, -279.4972802982216535, -337.3663333898606993 ) ) ;
#83463=CARTESIAN_POINT ( 'NONE',  ( -34.77913880771958333, -296.3236811867578808, -194.3752002295109662 ) ) ;
#83464=CARTESIAN_POINT ( 'NONE',  ( -95.61650295640320962, -279.8994201434853153, -317.8583741363235049 ) ) ;
#83466=CARTESIAN_POINT ( 'NONE',  ( -108.8537920578055491, -286.1590073307670536, -294.7606037356579805 ) ) ;
#83469=CARTESIAN_POINT ( 'NONE',  ( 24.83329132087108349, -284.9835232049495062, -228.3262140529449766 ) ) ;
#83471=CARTESIAN_POINT ( 'NONE',  ( -109.5354678547003573, -295.1724987090038326, -283.6667710372168472 ) ) ;
#83472=CARTESIAN_POINT ( 'NONE',  ( -70.54588100114629867, -287.6342580605751209, -336.7706046577903294 ) ) ;
#83473=CARTESIAN_POINT ( 'NONE',  ( 60.10016229265469434, 49.69813606028536412, -316.8989054076328671 ) ) ;
#83474=CARTESIAN_POINT ( 'NONE',  ( -112.3856634378736032, -294.5377763325769820, -271.4678884910789520 ) ) ;
#83475=CARTESIAN_POINT ( 'NONE',  ( -52.02077281295309064, -284.3475746318123925, -195.4257635182382558 ) ) ;
#83476=CARTESIAN_POINT ( 'NONE',  ( 33.73536812890394998, -283.4119494634100533, -290.2229100550771932 ) ) ;
#83477=CARTESIAN_POINT ( 'NONE',  ( -63.58337598135658908, -281.6294238540601214, -341.6727471993660856 ) ) ;
#83478=CARTESIAN_POINT ( 'NONE',  ( -94.10428572898682376, -289.9028999145141938, -316.2632843355752925 ) ) ;
#83479=CARTESIAN_POINT ( 'NONE',  ( -96.89312957719243968, -280.5775870478598790, -227.1291602576011712 ) ) ;
#83480=CARTESIAN_POINT ( 'NONE',  ( 7.232630231837879009, -281.4799188724474561, -212.2821068637000508 ) ) ;
#83481=CARTESIAN_POINT ( 'NONE',  ( 2.335988668896574971, -290.5036862728474603, -334.4854965381022680 ) ) ;
#83483=CARTESIAN_POINT ( 'NONE',  ( -101.2085470588424272, -273.1198838868033363, -227.2542674860649470 ) ) ;
#83484=CARTESIAN_POINT ( 'NONE',  ( -91.97995764589691703, -293.2473193901424793, -219.4844929036364078 ) ) ;
#83486=CARTESIAN_POINT ( 'NONE',  ( -72.08107566293803359, -294.1233781216987495, -198.2974183793908196 ) ) ;
#83489=CARTESIAN_POINT ( 'NONE',  ( 24.54266787001388650, -274.1300837361697518, -313.1167648979428577 ) ) ;
#83491=CARTESIAN_POINT ( 'NONE',  ( -27.86771615180484218, -293.3337838255895917, -346.0226123158192877 ) ) ;
#83492=CARTESIAN_POINT ( 'NONE',  ( -92.78701748118989201, -296.7367470087901324, -222.7624144439384395 ) ) ;
#83493=CARTESIAN_POINT ( 'NONE',  ( 6.270381546870561706, -289.9683582228354908, -329.8275374989206057 ) ) ;
#83494=CARTESIAN_POINT ( 'NONE',  ( -42.98816216063917039, -284.8843999989980489, -344.2095388006447365 ) ) ;
#83495=CARTESIAN_POINT ( 'NONE',  ( -107.8306215674464568, -292.3554510102356403, -240.8667414716206849 ) ) ;
#83496=CARTESIAN_POINT ( 'NONE',  ( -64.23126705966906513, -293.0238351612961765, -198.6795392366130102 ) ) ;
#83497=CARTESIAN_POINT ( 'NONE',  ( -62.79874002224426732, -291.5446184517837764, -201.9437289332097407 ) ) ;
#83498=CARTESIAN_POINT ( 'NONE',  ( -107.4431108929004353, -286.8987710334055805, -243.7004192748076719 ) ) ;
#83499=CARTESIAN_POINT ( 'NONE',  ( -39.58938593284456431, -280.1913707393119353, -193.3808800750918522 ) ) ;
#83500=CARTESIAN_POINT ( 'NONE',  ( -110.9095010193052957, -294.4116173836607686, -287.6535395666318209 ) ) ;
#83501=CARTESIAN_POINT ( 'NONE',  ( 4.543917342797125336, -282.3373657984004694, -335.0352412674635616 ) ) ;
#83502=CARTESIAN_POINT ( 'NONE',  ( 34.79231427388593545, -277.6407318583409278, -287.9518260514425378 ) ) ;
#83503=CARTESIAN_POINT ( 'NONE',  ( -85.28047601435908120, -298.1948066931273615, -330.5268031993605859 ) ) ;
#83504=CARTESIAN_POINT ( 'NONE',  ( -110.2583065397283946, -276.4296316844952344, -290.9396016805934551 ) ) ;
#83507=CARTESIAN_POINT ( 'NONE',  ( -86.97523656896281352, -283.2729626921415047, -324.0447068728149702 ) ) ;
#83509=CARTESIAN_POINT ( 'NONE',  ( -42.41913721670286463, -281.1945235871316413, -193.9266470193877865 ) ) ;
#83510=CARTESIAN_POINT ( 'NONE',  ( 37.49295188953270497, -286.3956630625942239, -253.1973278739361604 ) ) ;
#83511=CARTESIAN_POINT ( 'NONE',  ( -49.88217404808551692, -293.6502793456660925, -197.3658772377385162 ) ) ;
#83512=CARTESIAN_POINT ( 'NONE',  ( -1.693978837971687801, -276.1166892704454199, -203.0136578687803137 ) ) ;
#83514=CARTESIAN_POINT ( 'NONE',  ( 28.67889689226771566, -277.3737587020327169, -309.0209038182451309 ) ) ;
#83515=CARTESIAN_POINT ( 'NONE',  ( 16.52972094407187242, -276.0923400715444700, -319.6430337401266115 ) ) ;
#83516=CARTESIAN_POINT ( 'NONE',  ( -110.9407071720953581, -298.3772169346628971, -283.9676526752120935 ) ) ;
#83517=CARTESIAN_POINT ( 'NONE',  ( -109.7975279541543046, -282.7929746636296500, -251.6479823908108244 ) ) ;
#83519=CARTESIAN_POINT ( 'NONE',  ( -39.20692436760563027, -291.6960974933989519, -193.3918309911692575 ) ) ;
#83520=CARTESIAN_POINT ( 'NONE',  ( 36.37570793743105213, -289.3962956810174774, -289.6531931783655978 ) ) ;
#83521=CARTESIAN_POINT ( 'NONE',  ( 18.72182795199518424, -291.8042567305818693, -223.1265237357260673 ) ) ;
#83523=CARTESIAN_POINT ( 'NONE',  ( -79.25592021465617165, -290.0735515596680898, -206.4088780873719600 ) ) ;
#83524=CARTESIAN_POINT ( 'NONE',  ( -4.819850047954069794, -292.1593566701213263, -204.9681651676269212 ) ) ;
#83526=CARTESIAN_POINT ( 'NONE',  ( -43.14513492355533941, -290.2034799911207301, -346.8321102238632534 ) ) ;
#83527=CARTESIAN_POINT ( 'NONE',  ( -85.50130918654589607, -279.6973397814891769, -215.4726898576277563 ) ) ;
#83528=CARTESIAN_POINT ( 'NONE',  ( -114.0287313637569611, -295.4821416439342556, -269.5918656632948682 ) ) ;
#83529=CARTESIAN_POINT ( 'NONE',  ( -21.01370799430131697, -286.9077985944710463, -195.2165276307016768 ) ) ;
#83530=CARTESIAN_POINT ( 'NONE',  ( 39.33319754247998645, -287.7927842176408149, -262.9550734836485617 ) ) ;
#83531=CARTESIAN_POINT ( 'NONE',  ( -109.6337561475086204, -285.0211776174291458, -260.0681046597024419 ) ) ;
#83532=CARTESIAN_POINT ( 'NONE',  ( 102.8821184830924267, 116.5732156867659342, -282.8887793008179870 ) ) ;
#83533=CARTESIAN_POINT ( 'NONE',  ( -78.94308665734938302, -207.6905716540671278, -356.1245641789462297 ) ) ;
#83534=CARTESIAN_POINT ( 'NONE',  ( 44.56609888530009300, 11.47358219897120080, -328.3762950272841294 ) ) ;
#83535=CARTESIAN_POINT ( 'NONE',  ( -8.898633777073184703, -273.6310117220890561, -202.9008987423906376 ) ) ;
#83536=CARTESIAN_POINT ( 'NONE',  ( 18.53513759638890690, -275.1444237426023847, -317.8164135808054311 ) ) ;
#83537=CARTESIAN_POINT ( 'NONE',  ( -112.8270871651255618, -296.2469278174632450, -255.4110798984995370 ) ) ;
#83538=CARTESIAN_POINT ( 'NONE',  ( 104.3072796027752673, 114.1787421069637105, -280.1511098027236812 ) ) ;
#83539=CARTESIAN_POINT ( 'NONE',  ( 34.26611105204779761, -273.8939975902330275, -243.4237897955941321 ) ) ;
#83540=CARTESIAN_POINT ( 'NONE',  ( -111.3558677489446183, -274.3479423682161382, -267.6218071371351925 ) ) ;
#83542=CARTESIAN_POINT ( 'NONE',  ( -3.551308916552529560, -299.4067538136396252, -193.5911544943717217 ) ) ;
#83543=CARTESIAN_POINT ( 'NONE',  ( -50.75661716430504811, -289.7203767828612513, -342.2322550546592765 ) ) ;
#83544=CARTESIAN_POINT ( 'NONE',  ( -114.1487856353897712, -297.4002016366695784, -266.7530796441062080 ) ) ;
#83545=CARTESIAN_POINT ( 'NONE',  ( -82.93915359280163102, -297.9395659979604716, -208.3239650866019588 ) ) ;
#83546=CARTESIAN_POINT ( 'NONE',  ( -80.15306037536085171, -295.8169075192104174, -329.4896850061484201 ) ) ;
#83548=CARTESIAN_POINT ( 'NONE',  ( -31.53604330725120164, -278.8996815272684557, -345.7493916958144951 ) ) ;
#83550=CARTESIAN_POINT ( 'NONE',  ( 23.70231203714039836, -280.4343936723595334, -223.5084555303059233 ) ) ;
#83551=UNCERTAINTY_MEASURE_WITH_UNIT (LENGTH_MEASURE( 1.000000000000000082E-05 ), #64964, 'distance_accuracy_value', 'NONE');
#83552=CARTESIAN_POINT ( 'NONE',  ( -89.24414438008285799, -278.7456658904580422, -322.1007552218759429 ) ) ;
#83553=CARTESIAN_POINT ( 'NONE',  ( -38.50664539732039060, -278.8267058698347682, -346.3388576137431301 ) ) ;
#83554=CARTESIAN_POINT ( 'NONE',  ( -73.33391107725348945, -275.5471112762936627, -336.5797862244453427 ) ) ;
#83555=CARTESIAN_POINT ( 'NONE',  ( -107.2572525056515218, -273.3271543561581325, -248.9791829637545106 ) ) ;
#83556=CARTESIAN_POINT ( 'NONE',  ( -63.27021795266994530, -296.2824949836247583, -201.4371405066596594 ) ) ;
#83558=CARTESIAN_POINT ( 'NONE',  ( -107.1159935047156324, -278.4325508829217597, -291.9907512978328441 ) ) ;
#83559=CARTESIAN_POINT ( 'NONE',  ( -23.41823235009659143, -287.5626910537846470, -345.6441027961407713 ) ) ;
#83560=CARTESIAN_POINT ( 'NONE',  ( -90.76284863589798135, -275.2946102174046246, -217.7191049127725648 ) ) ;
#83562=CARTESIAN_POINT ( 'NONE',  ( -109.5801722296861556, -289.5957942488715844, -282.0246663936416667 ) ) ;
#83563=CARTESIAN_POINT ( 'NONE',  ( -114.0495132143409620, -283.9772938462530192, -264.2480709591835648 ) ) ;
#83564=CARTESIAN_POINT ( 'NONE',  ( 20.96561177439674495, -280.4258233502402504, -315.9487412495511194 ) ) ;
#83565=CARTESIAN_POINT ( 'NONE',  ( 36.01481182132828707, -280.2114044299391935, -276.8207810982214596 ) ) ;
#83566=CARTESIAN_POINT ( 'NONE',  ( -104.7798596275713834, -283.0508188132958480, -238.7206201930535485 ) ) ;
#83567=CARTESIAN_POINT ( 'NONE',  ( -16.90200753173384385, -288.3161387804996139, -198.1466682588884112 ) ) ;
#83568=CARTESIAN_POINT ( 'NONE',  ( -96.73600627050431910, -280.3574260664447024, -227.2398134632963718 ) ) ;
#83571=CARTESIAN_POINT ( 'NONE',  ( -22.61216942323112278, -294.2407228081135031, -196.7688180487071179 ) ) ;
#83572=CARTESIAN_POINT ( 'NONE',  ( -113.3713618042508671, -276.7766952380807766, -271.5696119474641250 ) ) ;
#83574=CARTESIAN_POINT ( 'NONE',  ( -94.85080901949508814, -285.8844174751034188, -318.7827891345715443 ) ) ;
#83577=CARTESIAN_POINT ( 'NONE',  ( -72.48206884650126369, -291.4336579165063199, -337.2670659464135383 ) ) ;
#83579=CARTESIAN_POINT ( 'NONE',  ( -112.2279753225190149, -294.4881089321660284, -275.3361550871782129 ) ) ;
#83580=CARTESIAN_POINT ( 'NONE',  ( 5.099023081603529128, -285.8070168476255617, -206.2435135136128395 ) ) ;
#83581=CARTESIAN_POINT ( 'NONE',  ( -68.11641715727034807, -290.0410410176143046, -203.2699872277709403 ) ) ;
#83583=CARTESIAN_POINT ( 'NONE',  ( 22.86023606935548358, -274.8219652345104009, -312.6025875795114644 ) ) ;
#83584=CARTESIAN_POINT ( 'NONE',  ( -50.71661875223671245, -293.3643875934328094, -343.3815057487315130 ) ) ;
#83586=CARTESIAN_POINT ( 'NONE',  ( -37.77152332136167701, -290.5267452074634775, -194.0556594118756095 ) ) ;
#83587=CARTESIAN_POINT ( 'NONE',  ( -88.26104537463086785, -286.9245651406856723, -216.9414521880127040 ) ) ;
#83588=CARTESIAN_POINT ( 'NONE',  ( 25.00723104401543750, -286.3747244374912952, -313.8862593594518557 ) ) ;
#83590=CARTESIAN_POINT ( 'NONE',  ( -110.4560286155236071, -285.8624637120027501, -279.1465748536348883 ) ) ;
#83592=CARTESIAN_POINT ( 'NONE',  ( -9.441252023900927881, -287.2291755239171493, -202.7149949180676174 ) ) ;
#83593=CARTESIAN_POINT ( 'NONE',  ( 37.22056660734074285, -295.3882464338495311, -259.1088065173165660 ) ) ;
#83594=CARTESIAN_POINT ( 'NONE',  ( -102.3790337418371763, -276.1202220280419510, -308.9275197025054354 ) ) ;
#83595=CARTESIAN_POINT ( 'NONE',  ( 39.11710122699075498, -276.0027742400349666, -279.7411067331673848 ) ) ;
#83596=CARTESIAN_POINT ( 'NONE',  ( -22.45314311166790588, -290.3210391183087609, -196.2291638266372331 ) ) ;
#83597=CARTESIAN_POINT ( 'NONE',  ( -67.36245925523701317, -279.6691571329307635, -199.4544608802166294 ) ) ;
#83598=CARTESIAN_POINT ( 'NONE',  ( -106.4760059060146489, -298.1632874237901660, -298.5088455074348985 ) ) ;
#83601=CARTESIAN_POINT ( 'NONE',  ( -109.4845510343781143, -276.9187973830696592, -252.8604166639343305 ) ) ;
#83603=CARTESIAN_POINT ( 'NONE',  ( 36.68946876235337839, -279.7073047893435387, -282.4572760389032169 ) ) ;
#83606=CARTESIAN_POINT ( 'NONE',  ( 6.849372451248299853, -273.1209173928744463, -208.0880875547902065 ) ) ;
#83607=CARTESIAN_POINT ( 'NONE',  ( 20.24760536984477000, -295.7158373115918266, -316.3614508254897260 ) ) ;
#83609=CARTESIAN_POINT ( 'NONE',  ( 35.88466650688650361, -280.1850321800189931, -247.5709503830718461 ) ) ;
#83610=CARTESIAN_POINT ( 'NONE',  ( -90.57003437736362628, -296.7704952303038795, -320.7347617401772482 ) ) ;
#83611=CARTESIAN_POINT ( 'NONE',  ( -70.53035978945197826, -298.9388355138526663, -201.4277360464224955 ) ) ;
#83612=CARTESIAN_POINT ( 'NONE',  ( -33.80998169044987378, -297.9308959821268559, -197.3612213806951843 ) ) ;
#83613=CARTESIAN_POINT ( 'NONE',  ( -55.52113752425723447, -293.8183571015531470, -197.5977432556503572 ) ) ;
#83614=CARTESIAN_POINT ( 'NONE',  ( -114.3548223872009260, -284.6876880671820231, -272.8513511617020981 ) ) ;
#83615=CARTESIAN_POINT ( 'NONE',  ( 0.4106575901258024408, -274.6947651974198266, -336.1097712475500430 ) ) ;
#83616=CARTESIAN_POINT ( 'NONE',  ( 21.48764901255395543, -288.0547746324221521, -320.0411711650548341 ) ) ;
#83617=CARTESIAN_POINT ( 'NONE',  ( 22.93677463692982244, -287.1885722299908821, -311.9754517053271456 ) ) ;
#83618=CARTESIAN_POINT ( 'NONE',  ( -93.20417831708374479, -289.2489799202384120, -220.3172953790736699 ) ) ;
#83619=ORIENTED_EDGE ( 'NONE', *, *, #85455, .T. ) ;
#83620=CARTESIAN_POINT ( 'NONE',  ( 84.09003387609358526, 83.72762891241104910, -302.5758382668069544 ) ) ;
#83621=CARTESIAN_POINT ( 'NONE',  ( 14.12228742805320536, -287.8127915613035839, -322.2209909714188711 ) ) ;
#83623=CARTESIAN_POINT ( 'NONE',  ( -108.0058390277665268, -285.1089571944567069, -300.4870462044021906 ) ) ;
#83624=CARTESIAN_POINT ( 'NONE',  ( 20.21025720406927562, -291.9207381929551275, -219.5417231869045622 ) ) ;
#83625=CARTESIAN_POINT ( 'NONE',  ( -1.529620915453896890, -282.1190008418298589, -203.1009113272673972 ) ) ;
#83626=CARTESIAN_POINT ( 'NONE',  ( 25.86368855657732269, -282.2940102327014529, -227.1598092541180733 ) ) ;
#83627=CARTESIAN_POINT ( 'NONE',  ( -100.4021996277868851, -283.8807591070132048, -307.1357479241078181 ) ) ;
#83628=CARTESIAN_POINT ( 'NONE',  ( 20.74635420978414047, -278.2062920974549911, -317.8237358363423937 ) ) ;
#83629=CARTESIAN_POINT ( 'NONE',  ( -65.54200561698550587, -297.6935812576494982, -198.6539872572283230 ) ) ;
#83630=CARTESIAN_POINT ( 'NONE',  ( -97.09991869523867081, -287.9580211839782464, -315.1127845529509273 ) ) ;
#83631=CARTESIAN_POINT ( 'NONE',  ( -79.06826775116425665, -272.2706420845412367, -209.9170738562476402 ) ) ;
#83635=CARTESIAN_POINT ( 'NONE',  ( -92.60639422852541713, -287.1733562218302609, -220.4142353466645261 ) ) ;
#83636=CARTESIAN_POINT ( 'NONE',  ( 23.79093163603620198, -295.2512064732600834, -316.6676385211700904 ) ) ;
#83637=CARTESIAN_POINT ( 'NONE',  ( -65.13965640441421101, -286.3306198861232019, -202.6968311293901763 ) ) ;
#83638=CARTESIAN_POINT ( 'NONE',  ( -9.308939621169331602, -275.7532582758374247, -341.8242871772670242 ) ) ;
#83639=CARTESIAN_POINT ( 'NONE',  ( -64.36076891912699693, -292.3601814055583077, -198.3099978050392167 ) ) ;
#83640=CARTESIAN_POINT ( 'NONE',  ( -69.25068512362842910, -283.7764786004359507, -201.6292855902406700 ) ) ;
#83641=CARTESIAN_POINT ( 'NONE',  ( -77.16196030773112113, -291.8674319771969294, -204.4202724241321789 ) ) ;
#83642=CARTESIAN_POINT ( 'NONE',  ( -63.82460531587253172, -289.7403612548397973, -338.4648817304469048 ) ) ;
#83643=FACE_OUTER_BOUND ( 'NONE', #62736, .T. ) ;
#83646=CARTESIAN_POINT ( 'NONE',  ( 189.2201263495670958, 268.0219113037794614, -137.5448743359141019 ) ) ;
#83647=CARTESIAN_POINT ( 'NONE',  ( -94.79979063882947798, -285.3869565282979011, -320.5734231346647221 ) ) ;
#83648=CARTESIAN_POINT ( 'NONE',  ( -69.85430415644619018, -283.1237833571632336, -202.7746430608542312 ) ) ;
#83650=CARTESIAN_POINT ( 'NONE',  ( 22.83066784913029679, -281.0536917245429436, -312.2360771581774088 ) ) ;
#83651=CARTESIAN_POINT ( 'NONE',  ( 32.99872845308576075, -275.6181197124072355, -301.6336042677241949 ) ) ;
#83652=CARTESIAN_POINT ( 'NONE',  ( -107.2355265971909546, -280.9023202287054346, -243.4785825081016810 ) ) ;
#83653=CARTESIAN_POINT ( 'NONE',  ( -110.6140932004204842, -273.3870535845430823, -283.9357899037859170 ) ) ;
#83654=CARTESIAN_POINT ( 'NONE',  ( 37.67965657171717453, -279.9440781558708409, -255.8558660642179632 ) ) ;
#83656=CARTESIAN_POINT ( 'NONE',  ( -92.72503140558073653, -283.2739396131223657, -220.2398861061249704 ) ) ;
#83657=CARTESIAN_POINT ( 'NONE',  ( -110.6296720769561972, -274.6593297104210478, -250.9460721357923489 ) ) ;
#83659=CARTESIAN_POINT ( 'NONE',  ( -61.02719283052873323, -295.8602783437192443, -339.5304785176875839 ) ) ;
#83661=CARTESIAN_POINT ( 'NONE',  ( -33.46579123389754074, -290.7867488611997260, -196.9576646622759029 ) ) ;
#83662=CARTESIAN_POINT ( 'NONE',  ( 27.56725041205460514, -276.7457894615187115, -311.6928796239213284 ) ) ;
#83663=CARTESIAN_POINT ( 'NONE',  ( -6.528980864048501864, -274.4684564035028416, -204.1827504327639531 ) ) ;
#83664=CARTESIAN_POINT ( 'NONE',  ( 14.66342823393550532, -275.2609211811513319, -326.7979036708752005 ) ) ;
#83666=CARTESIAN_POINT ( 'NONE',  ( -107.3513634428434784, -270.9033725294536907, -243.3185114834425065 ) ) ;
#83671=CARTESIAN_POINT ( 'NONE',  ( -23.99578925850525835, -283.9573320297236023, -342.4451851249907008 ) ) ;
#83672=CARTESIAN_POINT ( 'NONE',  ( 35.51362451769220741, -283.5888259353502008, -292.1311024125701010 ) ) ;
#83673=CARTESIAN_POINT ( 'NONE',  ( -103.1079902031413269, -283.4678692589171760, -302.3942872770173267 ) ) ;
#83674=CARTESIAN_POINT ( 'NONE',  ( 19.78808432388189686, -274.6065859171814623, -317.0996303155948226 ) ) ;
#83675=CARTESIAN_POINT ( 'NONE',  ( 10.72623435313587059, -284.2403092013405512, -327.0002776758514642 ) ) ;
#83676=CARTESIAN_POINT ( 'NONE',  ( -109.4471449020585538, -276.8331981486666109, -285.5766557105600327 ) ) ;
#83678=CARTESIAN_POINT ( 'NONE',  ( -27.26122141817058164, -275.2628131234124567, -197.6972645889283626 ) ) ;
#83680=CARTESIAN_POINT ( 'NONE',  ( -96.69923366365264883, -280.0119705313902614, -221.5467817715656338 ) ) ;
#83684=CARTESIAN_POINT ( 'NONE',  ( -62.80890407608294623, -287.5845191447024831, -199.0047797732487425 ) ) ;
#83685=CARTESIAN_POINT ( 'NONE',  ( -23.49827999087680652, -294.0679488439579927, -342.2526671583277107 ) ) ;
#83686=CARTESIAN_POINT ( 'NONE',  ( -114.2666556469257131, -289.9259366616903435, -268.3490902008105081 ) ) ;
#83687=CARTESIAN_POINT ( 'NONE',  ( 20.31856066047237519, -285.1447471103097655, -223.9377082656914126 ) ) ;
#83688=CARTESIAN_POINT ( 'NONE',  ( 36.27028063202638464, -286.1000840102910843, -268.3140329276992588 ) ) ;
#83689=CARTESIAN_POINT ( 'NONE',  ( -110.9788537831871054, -288.8889729717097339, -262.9083591717460990 ) ) ;
#83690=CARTESIAN_POINT ( 'NONE',  ( -98.44609493244351484, -286.3186188348701080, -229.6993000141757761 ) ) ;
#83691=CARTESIAN_POINT ( 'NONE',  ( -39.92038152832244435, -275.0843633331755314, -345.3295050678155462 ) ) ;
#83692=CARTESIAN_POINT ( 'NONE',  ( -46.39007835770571830, -284.3390262087961560, -194.7002478726284096 ) ) ;
#83693=CARTESIAN_POINT ( 'NONE',  ( -29.35235599798215134, -300.1523195474867407, -195.3583854697037054 ) ) ;
#83694=CARTESIAN_POINT ( 'NONE',  ( 36.86089110167503691, -285.7097769764948225, -282.6770705386612690 ) ) ;
#83695=CARTESIAN_POINT ( 'NONE',  ( 17.23016830472284155, -281.7968823512113659, -221.5213839106548903 ) ) ;
#83696=CARTESIAN_POINT ( 'NONE',  ( -94.05783607469211915, -291.8692315460991722, -319.6896933938890015 ) ) ;
#83699=CARTESIAN_POINT ( 'NONE',  ( -98.82230144032514829, -297.8783128380003404, -314.3747118235620519 ) ) ;
#83700=CARTESIAN_POINT ( 'NONE',  ( 6.101821325143905739, -278.6415284164199306, -209.2247042026039594 ) ) ;
#83701=CARTESIAN_POINT ( 'NONE',  ( -53.34568327821199318, -291.0492293343397705, -195.1533504221171427 ) ) ;
#83702=CARTESIAN_POINT ( 'NONE',  ( -95.06443740709715939, -295.5943986711673119, -224.3771423080110878 ) ) ;
#83703=CARTESIAN_POINT ( 'NONE',  ( 29.75791416870868389, -280.6394854804789247, -300.4674218182362893 ) ) ;
#83704=CARTESIAN_POINT ( 'NONE',  ( 34.25159369914924667, -273.3654809044871854, -249.7876352249365937 ) ) ;
#83705=CARTESIAN_POINT ( 'NONE',  ( 22.19443561198040982, -294.2682909721281703, -227.2503748406092257 ) ) ;
#83706=CARTESIAN_POINT ( 'NONE',  ( 31.98288692825981272, -296.4805209788416391, -303.7098442033570223 ) ) ;
#83707=CARTESIAN_POINT ( 'NONE',  ( -112.2046667397903263, -295.2193192331176306, -255.5209238969743808 ) ) ;
#83708=CARTESIAN_POINT ( 'NONE',  ( 23.20775597478778352, -292.4118531398285086, -316.2712190717501244 ) ) ;
#83710=CARTESIAN_POINT ( 'NONE',  ( -110.3720588842078740, -291.8589733440334157, -279.4132788741173954 ) ) ;
#83713=CARTESIAN_POINT ( 'NONE',  ( -57.70967943973177228, -292.5853005307996568, -200.0390167523388527 ) ) ;
#83715=CARTESIAN_POINT ( 'NONE',  ( -105.5282640988716736, -282.1524235935357297, -302.4391368366162851 ) ) ;
#83716=CARTESIAN_POINT ( 'NONE',  ( 33.44606184527689408, -293.7875351576128651, -288.1962730086082729 ) ) ;
#83717=VECTOR ( 'NONE', #7875, 1000.000000000000000 ) ;
#83718=CARTESIAN_POINT ( 'NONE',  ( 39.18277429408395562, -281.4394552767052460, -261.3499659589428461 ) ) ;
#83719=CARTESIAN_POINT ( 'NONE',  ( -111.0889411197778855, -283.9413196168746936, -292.4769865206196755 ) ) ;
#83720=CARTESIAN_POINT ( 'NONE',  ( -40.04936459777392344, -287.0859725935235929, -345.1962801798966893 ) ) ;
#83722=CARTESIAN_POINT ( 'NONE',  ( 10.40439963802415413, -279.1770969573357775, -210.7701246941907129 ) ) ;
#83724=CARTESIAN_POINT ( 'NONE',  ( 0.5545326242041785925, -287.4800480722837506, -337.0947171187447111 ) ) ;
#83726=CARTESIAN_POINT ( 'NONE',  ( 34.99664873470414506, -294.9615744125441665, -255.7459306463501605 ) ) ;
#83727=CARTESIAN_POINT ( 'NONE',  ( 27.16124974261197522, -277.5195238057606844, -311.4226089470499232 ) ) ;
#83728=CARTESIAN_POINT ( 'NONE',  ( -89.48570549627913806, -278.9592817926890689, -219.1710697254665945 ) ) ;
#83729=CARTESIAN_POINT ( 'NONE',  ( 13.27688018601567776, -292.9041851990604073, -212.3373355181988416 ) ) ;
#83731=CARTESIAN_POINT ( 'NONE',  ( -71.11741497043608717, -281.5743188162936690, -337.9519109115691435 ) ) ;
#83733=CARTESIAN_POINT ( 'NONE',  ( 20.37571500980241623, -291.9773247881270777, -225.2618984494971244 ) ) ;
#83734=CARTESIAN_POINT ( 'NONE',  ( -107.9589445449695688, -294.8793984392997913, -245.0983897371746707 ) ) ;
#83738=CARTESIAN_POINT ( 'NONE',  ( -18.21041960237902302, -294.3064864114428474, -340.8734044787660764 ) ) ;
#83739=DIRECTION ( 'NONE',  ( 1.000000000000000000, 0.000000000000000000, 0.000000000000000000 ) ) ;
#83740=CARTESIAN_POINT ( 'NONE',  ( -37.30987171927208834, -283.5523547857346784, -200.3611179825600459 ) ) ;
#83741=CARTESIAN_POINT ( 'NONE',  ( -34.75720343727335404, -297.1425210244456707, -193.5968116746220460 ) ) ;
#83742=CARTESIAN_POINT ( 'NONE',  ( 10.06882940760500134, -278.8368577378015516, -211.1960796480762497 ) ) ;
#83743=CARTESIAN_POINT ( 'NONE',  ( -40.81098369611125065, -287.3246733916650442, -193.8811083699249309 ) ) ;
#83744=CARTESIAN_POINT ( 'NONE',  ( 22.74869363240472708, -287.9630191484949933, -311.8336583687811867 ) ) ;
#83745=CARTESIAN_POINT ( 'NONE',  ( -96.63949041376348248, -279.4645187621603100, -314.1370317710530458 ) ) ;
#83746=CARTESIAN_POINT ( 'NONE',  ( -112.0302531516438194, -294.5580413597796792, -271.4627843704465135 ) ) ;
#83747=CARTESIAN_POINT ( 'NONE',  ( -94.40905279170833353, -298.9714244982031346, -223.2108184744342054 ) ) ;
#83749=CARTESIAN_POINT ( 'NONE',  ( -69.43884146103015098, -276.2791051981377564, -336.3818797203672375 ) ) ;
#83751=CARTESIAN_POINT ( 'NONE',  ( -36.18052107874536460, -297.7330388629878826, -193.3823253170526755 ) ) ;
#83752=CARTESIAN_POINT ( 'NONE',  ( -53.70166852880146990, -291.1838859353031808, -342.9811264430320534 ) ) ;
#83753=CARTESIAN_POINT ( 'NONE',  ( 12.88399548592787980, -295.9652470364154055, -327.7357191750959942 ) ) ;
#83754=CARTESIAN_POINT ( 'NONE',  ( 202.8417115650362064, 291.9636489450775798, -53.99999999997881872 ) ) ;
#83755=CARTESIAN_POINT ( 'NONE',  ( -106.6705898391738998, -291.5110177175811828, -247.1792776850786595 ) ) ;
#83757=CARTESIAN_POINT ( 'NONE',  ( -103.0242062971173169, -296.6806908124781899, -310.3501310955515464 ) ) ;
#83758=CARTESIAN_POINT ( 'NONE',  ( -94.70988034397520039, -289.3711456539789992, -220.8519292617993131 ) ) ;
#83759=CARTESIAN_POINT ( 'NONE',  ( -105.2369621212111070, -297.3556261521179067, -233.9716225015516216 ) ) ;
#83762=CARTESIAN_POINT ( 'NONE',  ( -72.83405174706639684, -291.0336904919063841, -337.9257268898228972 ) ) ;
#83763=CARTESIAN_POINT ( 'NONE',  ( -111.2869819898779866, -293.6237833571632905, -305.9350535429201159 ) ) ;
#83764=CARTESIAN_POINT ( 'NONE',  ( -49.74998625019737375, -287.8938299353961838, -196.5108785158396358 ) ) ;
#83765=CARTESIAN_POINT ( 'NONE',  ( -43.59976985966797969, -284.5494196383076542, -194.1541935519939841 ) ) ;
#83766=CARTESIAN_POINT ( 'NONE',  ( -65.22891867520753806, -271.6867263491052427, -200.9042931272572901 ) ) ;
#83767=CARTESIAN_POINT ( 'NONE',  ( -29.86915946427574653, -276.0676374165018387, -196.2971231313207170 ) ) ;
#83768=CARTESIAN_POINT ( 'NONE',  ( -87.72159621072766811, -287.8418205613744476, -325.2323475115753126 ) ) ;
#83769=CARTESIAN_POINT ( 'NONE',  ( -53.83883943083342416, -279.1219846508457181, -344.3618179644143424 ) ) ;
#83771=CARTESIAN_POINT ( 'NONE',  ( -69.74029361473012045, -279.6132566577916236, -204.9306757305529914 ) ) ;
#83772=CARTESIAN_POINT ( 'NONE',  ( -4.294075338245559870, -279.8482884150208179, -205.1417840895167046 ) ) ;
#83773=CARTESIAN_POINT ( 'NONE',  ( -9.311941745198748066, -277.7738555204592217, -341.7461665208114141 ) ) ;
#83774=CARTESIAN_POINT ( 'NONE',  ( 38.78994780296864064, -280.2345737860297845, -261.4116726539747333 ) ) ;
#83775=CARTESIAN_POINT ( 'NONE',  ( 191.8115894054295723, 277.2456744639775934, -124.3514335590991351 ) ) ;
#83776=CARTESIAN_POINT ( 'NONE',  ( 29.73608067869177773, -276.0067991666836633, -232.9236822774168729 ) ) ;
#83778=CARTESIAN_POINT ( 'NONE',  ( -63.33923436811479490, -275.2395878527539139, -198.6196657700898243 ) ) ;
#83779=CARTESIAN_POINT ( 'NONE',  ( 34.45848030099739390, -278.0519495502701375, -270.3284710469131937 ) ) ;
#83783=CARTESIAN_POINT ( 'NONE',  ( 15.24168261024363780, -287.8963673640045613, -219.2806527016049074 ) ) ;
#83784=CARTESIAN_POINT ( 'NONE',  ( 28.04335104957394265, -289.8233730422027747, -309.0750572626094481 ) ) ;
#83785=CARTESIAN_POINT ( 'NONE',  ( -108.8084738454747935, -290.1032771662269170, -254.9860432518425455 ) ) ;
#83786=CARTESIAN_POINT ( 'NONE',  ( 7.513147032221117350, -286.1532649965426458, -207.7849405391121707 ) ) ;
#83788=CARTESIAN_POINT ( 'NONE',  ( 3.819701787755762634, -280.8880928513618755, -331.6779581204693272 ) ) ;
#83789=CARTESIAN_POINT ( 'NONE',  ( 36.21683723239629416, -289.2779869966798287, -259.9861718491330294 ) ) ;
#83790=CARTESIAN_POINT ( 'NONE',  ( -23.95839367581954349, -281.3579571241756980, -342.8290064511082846 ) ) ;
#83791=CARTESIAN_POINT ( 'NONE',  ( -59.90082660569489548, -281.0689601138114995, -200.3622609926799782 ) ) ;
#83793=CARTESIAN_POINT ( 'NONE',  ( -27.00661709502031371, -277.4095408039930248, -342.6879767574355924 ) ) ;
#83794=CARTESIAN_POINT ( 'NONE',  ( -113.9929757534116703, -289.3364193224434757, -271.2089663723333501 ) ) ;
#83795=CARTESIAN_POINT ( 'NONE',  ( -93.80803464921662282, -286.0666591789097311, -218.1706349736725770 ) ) ;
#83796=CARTESIAN_POINT ( 'NONE',  ( -15.43698499778952637, -286.8205061370775866, -196.5513793784771508 ) ) ;
#83797=CARTESIAN_POINT ( 'NONE',  ( 33.75990650994296516, -281.5006428796340856, -253.8214221561174213 ) ) ;
#83800=CARTESIAN_POINT ( 'NONE',  ( -108.6941563864936739, -292.0839460738015418, -295.9945958192292323 ) ) ;
#83802=CARTESIAN_POINT ( 'NONE',  ( -8.680324368668214774, -291.1043027850038243, -199.4257684546907967 ) ) ;
#83804=CARTESIAN_POINT ( 'NONE',  ( 31.34313224059402714, -274.2731225449401791, -244.9484784058903131 ) ) ;
#83805=CARTESIAN_POINT ( 'NONE',  ( -37.69684412098850856, -294.4050444960540176, -347.2714263640753529 ) ) ;
#83806=CARTESIAN_POINT ( 'NONE',  ( -33.45266957547072906, -290.5818340151796519, -196.7578611941518147 ) ) ;
#83807=B_SPLINE_CURVE_WITH_KNOTS ( 'NONE', 3,
 ( #54873, #83754, #19832, #26939, #76663, #47765, #62472, #41105, #11790, #91314, #48229, #12261, #91788, #55827, #50590, #43021, #58179, #87021, #7045, #93657, #64833, #21714, #21238, #14156, #78081, #28817, #14619, #34978, #64377, #56788 ),
 .UNSPECIFIED., .F., .F.,
 ( 4, 2, 2, 2, 2, 2, 2, 2, 2, 2, 2, 2, 2, 2, 4 ),
 ( 0.000000000000000000, 0.0003908071623920878011, 0.0007816143247841756021, 0.001172421487176263403, 0.001563228649568351204, 0.002344842974352409279, 0.003126457299136467353, 0.003517264461528496391, 0.003908071623920524561, 0.004298878786312553164, 0.004689685948704582635, 0.005080493111096611239, 0.005471300273488639843, 0.005862107435880668446, 0.006252914598272697050 ),
 .UNSPECIFIED. ) ;
#83808=CARTESIAN_POINT ( 'NONE',  ( 13.02831800923248196, -292.5772533925004950, -324.6608108447870222 ) ) ;
#83809=CARTESIAN_POINT ( 'NONE',  ( -42.67754315469100135, -290.3259037179245752, -343.6148609239481857 ) ) ;
#83811=CARTESIAN_POINT ( 'NONE',  ( -56.74817810252171313, -291.3023910043950764, -342.8605539464959975 ) ) ;
#83812=CARTESIAN_POINT ( 'NONE',  ( -17.09535120299540978, -290.3127891164427865, -197.9724878048348558 ) ) ;
#83813=CARTESIAN_POINT ( 'NONE',  ( -2.273194515521165915, -296.5886059270989108, -336.7140916198875402 ) ) ;
#83814=CARTESIAN_POINT ( 'NONE',  ( -93.44304845314134411, -286.1597395155926620, -223.2862078405397881 ) ) ;
#83815=CARTESIAN_POINT ( 'NONE',  ( 22.58319217484764962, -296.1715466622551958, -315.7377167139565586 ) ) ;
#83816=CARTESIAN_POINT ( 'NONE',  ( -18.97579045949714782, -276.2671760878968712, -197.2244370412116439 ) ) ;
#83817=CARTESIAN_POINT ( 'NONE',  ( 10.26721067062497994, -275.2071967860114796, -330.4405094951238198 ) ) ;
#83819=CARTESIAN_POINT ( 'NONE',  ( -60.09050750711053013, -296.9619142118142463, -196.9119102270677217 ) ) ;
#83820=CARTESIAN_POINT ( 'NONE',  ( 34.56577036798375957, -274.0207605876565822, -287.9441185455851837 ) ) ;
#83821=CARTESIAN_POINT ( 'NONE',  ( -46.61201146376574656, -278.0135563864154165, -196.4484954042421805 ) ) ;
#83822=CARTESIAN_POINT ( 'NONE',  ( -32.68106511887405929, -275.3172437285948604, -197.0995713611181657 ) ) ;
#83823=CARTESIAN_POINT ( 'NONE',  ( 24.01763491674655526, -273.5167726619777682, -224.8238991709367838 ) ) ;
#83825=CARTESIAN_POINT ( 'NONE',  ( -98.58834061380095193, -297.9094438971769705, -230.2512916970663639 ) ) ;
#83827=CARTESIAN_POINT ( 'NONE',  ( -31.96975626570363360, -287.0049329891199932, -345.5760336180214836 ) ) ;
#83828=CARTESIAN_POINT ( 'NONE',  ( 19.00020729366106664, -274.7276416310530180, -223.9435623315623332 ) ) ;
#83829=CARTESIAN_POINT ( 'NONE',  ( 37.14441420239932512, -287.7964260024668874, -289.8756964291102918 ) ) ;
#83830=CARTESIAN_POINT ( 'NONE',  ( -38.92399575944390477, -288.7382159848314700, -347.3237104035712264 ) ) ;
#83831=CARTESIAN_POINT ( 'NONE',  ( -79.72127913954591349, -299.4627254855557226, -207.9896349472606971 ) ) ;
#83832=CARTESIAN_POINT ( 'NONE',  ( 30.03437436176456643, -291.9833174549009982, -303.0457475220817969 ) ) ;
#83833=CARTESIAN_POINT ( 'NONE',  ( 39.11634884246835497, -280.8514686251995727, -278.5115826226154923 ) ) ;
#83835=CARTESIAN_POINT ( 'NONE',  ( -7.849339673284405627, -278.4382835502037210, -201.3485681991572562 ) ) ;
#83837=CARTESIAN_POINT ( 'NONE',  ( 3.824691759201260144, -287.2795201743352322, -331.1879993357542276 ) ) ;
#83840=CARTESIAN_POINT ( 'NONE',  ( -99.95557580891174609, -289.1104353168259991, -228.9811999213561649 ) ) ;
#83841=CARTESIAN_POINT ( 'NONE',  ( -77.96920197815704512, -299.0966985934662148, -208.6892569347878066 ) ) ;
#83842=CARTESIAN_POINT ( 'NONE',  ( 31.86646859667727938, -283.3967016165115638, -302.8715703831161932 ) ) ;
#83843=CARTESIAN_POINT ( 'NONE',  ( -67.49561044007009514, -295.6788301438177768, -201.2465219436849964 ) ) ;
#83844=CARTESIAN_POINT ( 'NONE',  ( -67.78436866182518372, -283.4631951357076218, -336.7105259116786442 ) ) ;
#83845=CARTESIAN_POINT ( 'NONE',  ( -89.67384716508622944, -274.7212821661693738, -218.6240780282018648 ) ) ;
#83846=CARTESIAN_POINT ( 'NONE',  ( 35.53810108040848803, -276.2633003847489590, -263.3952242428138675 ) ) ;
#83848=CARTESIAN_POINT ( 'NONE',  ( -6.260484085812628940, -284.6439699216946337, -338.6176829535341994 ) ) ;
#83849=CARTESIAN_POINT ( 'NONE',  ( -102.2979889642521982, -271.9343324569760512, -236.2672922166874798 ) ) ;
#83851=CARTESIAN_POINT ( 'NONE',  ( 203.8614262746842201, 292.1666555297790069, -53.99999999998426858 ) ) ;
#83852=CARTESIAN_POINT ( 'NONE',  ( 38.35686161845388398, -293.5626672673940902, -284.5294341077632794 ) ) ;
#83853=CARTESIAN_POINT ( 'NONE',  ( -101.0254760614666054, -287.0578934632392247, -231.3238711511847328 ) ) ;
#83855=CARTESIAN_POINT ( 'NONE',  ( -119.3990491898856732, -276.0523547857346784, -270.3284710469131937 ) ) ;
#83856=CARTESIAN_POINT ( 'NONE',  ( -91.22311014998314249, -276.9914919884159872, -325.2165884382902732 ) ) ;
#83857=CARTESIAN_POINT ( 'NONE',  ( -82.39620480500543920, -288.0558237848652539, -331.8146127721043968 ) ) ;
#83858=CARTESIAN_POINT ( 'NONE',  ( -34.80345155149174019, -284.5398496307136043, -344.0232824041333970 ) ) ;
#83859=CARTESIAN_POINT ( 'NONE',  ( -9.587862702729344377, -278.4446481729323750, -338.9875442448548029 ) ) ;
#83860=CARTESIAN_POINT ( 'NONE',  ( -100.9187158449311568, -285.4141394514896319, -312.8419807037064402 ) ) ;
#83861=CARTESIAN_POINT ( 'NONE',  ( -36.20267861888595462, -281.8324784494802202, -343.7493536614051095 ) ) ;
#83862=CARTESIAN_POINT ( 'NONE',  ( -75.54592218180198415, -281.5430959747556585, -205.7612093468124215 ) ) ;
#83863=CARTESIAN_POINT ( 'NONE',  ( -38.35954047606500694, -274.2064022054048564, -193.3678455130843474 ) ) ;
#83864=CARTESIAN_POINT ( 'NONE',  ( -112.1756846062068149, -278.1579804633938693, -288.5512546450444802 ) ) ;
#83865=CARTESIAN_POINT ( 'NONE',  ( -50.70619976531285289, -297.1443490438134631, -343.5916057907743379 ) ) ;
#83868=CARTESIAN_POINT ( 'NONE',  ( -111.0668489603112192, -294.9136984068614993, -252.8995053916117683 ) ) ;
#83869=CARTESIAN_POINT ( 'NONE',  ( -5.044520822516396663, -276.1228047087200252, -335.9103585911216783 ) ) ;
#83870=CARTESIAN_POINT ( 'NONE',  ( -110.6615795018882977, -274.0392125733291664, -247.9940030099612329 ) ) ;
#83871=CARTESIAN_POINT ( 'NONE',  ( 36.64397342037946714, -289.3568447565173187, -273.7846549246695531 ) ) ;
#83873=CARTESIAN_POINT ( 'NONE',  ( -113.2515100987002370, -297.9741855112433768, -278.1334086309209965 ) ) ;
#83874=CARTESIAN_POINT ( 'NONE',  ( 4.025850345351407178, -295.7136128574110217, -334.8963196889432083 ) ) ;
#83875=CARTESIAN_POINT ( 'NONE',  ( -93.95986355746282470, -293.2324258621239892, -221.4283886615356778 ) ) ;
#83876=CARTESIAN_POINT ( 'NONE',  ( -13.70627317335899242, -278.3593261074861402, -199.3035480811219600 ) ) ;
#83877=CARTESIAN_POINT ( 'NONE',  ( -95.07249317763655938, -281.1245961154930342, -223.3667594332614499 ) ) ;
#83878=CARTESIAN_POINT ( 'NONE',  ( -111.6482811715772954, -294.6896229378324961, -265.9062095572635940 ) ) ;
#83879=CARTESIAN_POINT ( 'NONE',  ( -8.487003589242570811, -284.5390178380397970, -340.4718230149956071 ) ) ;
#83881=CARTESIAN_POINT ( 'NONE',  ( 26.64386745758308450, -285.9839204023475645, -234.4791109983779620 ) ) ;
#83882=CARTESIAN_POINT ( 'NONE',  ( 204.9738562182569979, 294.2969822784110079, -54.00000000001656275 ) ) ;
#83884=CARTESIAN_POINT ( 'NONE',  ( -94.97112907977204088, -284.8507503115266672, -225.4973504363775589 ) ) ;
#83886=CARTESIAN_POINT ( 'NONE',  ( 31.73703595662894728, -282.2013667048361754, -236.9280197314031682 ) ) ;
#83887=CARTESIAN_POINT ( 'NONE',  ( 51.75741359865251923, -299.6895210198656514, -197.2919279030197401 ) ) ;
#83888=CARTESIAN_POINT ( 'NONE',  ( -3.650083206593016438, -285.2818066339923462, -201.5507064699835382 ) ) ;
#83889=CARTESIAN_POINT ( 'NONE',  ( 3.686056364449620482, -281.5306953664110665, -205.4173405899487932 ) ) ;
#83890=CARTESIAN_POINT ( 'NONE',  ( -48.04088945800175736, -281.4386669150863440, -194.7548937926495967 ) ) ;
#83891=CARTESIAN_POINT ( 'NONE',  ( 33.54811550065814174, -282.2689621360876799, -300.5035687541375182 ) ) ;
#83892=CARTESIAN_POINT ( 'NONE',  ( -6.998514795304330072, -280.1237833571632336, -333.4427485647536855 ) ) ;
#83893=CARTESIAN_POINT ( 'NONE',  ( 195.0332379032363406, 278.6780395204132788, -125.9065900532892783 ) ) ;
#83894=ORIENTED_EDGE ( 'NONE', *, *, #44228, .F. ) ;
#83895=CARTESIAN_POINT ( 'NONE',  ( 18.64052951612779907, -276.8593582415225569, -220.6253460462095575 ) ) ;
#83896=CARTESIAN_POINT ( 'NONE',  ( 121.1092636158038403, 149.8039588042703087, -263.3851840300012555 ) ) ;
#83897=CARTESIAN_POINT ( 'NONE',  ( 15.06183806717322327, -280.3289999966299320, -323.5913329037326776 ) ) ;
#83898=CARTESIAN_POINT ( 'NONE',  ( -6.321397510775049966, -294.2141862193411725, -200.9804945590911416 ) ) ;
#83899=CARTESIAN_POINT ( 'NONE',  ( -31.60261734790722343, -294.3265146052269756, -343.2876046489433861 ) ) ;
#83900=CARTESIAN_POINT ( 'NONE',  ( -94.66126940491362518, -290.7565496858929350, -219.0386679121750149 ) ) ;
#83901=DIRECTION ( 'NONE',  ( -0.000000000000000000, 0.000000000000000000, 1.000000000000000000 ) ) ;
#83902=CARTESIAN_POINT ( 'NONE',  ( -86.03390104519358772, -294.2867982593514284, -329.2480932924295303 ) ) ;
#83903=CARTESIAN_POINT ( 'NONE',  ( 27.72629771473231131, -286.4228632554742831, -305.2921764237661932 ) ) ;
#83904=CARTESIAN_POINT ( 'NONE',  ( 15.20710713539905434, -296.1614482322070216, -322.8689835812512570 ) ) ;
#83905=CARTESIAN_POINT ( 'NONE',  ( -96.98478119270632192, -286.4640131319107468, -227.3984462652104810 ) ) ;
#83907=CARTESIAN_POINT ( 'NONE',  ( -58.88417168002998636, -292.7213230141007898, -196.6811198025568501 ) ) ;
#83908=CARTESIAN_POINT ( 'NONE',  ( -58.96036355089380265, -283.8317438056981246, -340.2041435065203814 ) ) ;
#83909=CARTESIAN_POINT ( 'NONE',  ( -83.95580386430142994, -294.4711059590339346, -331.2156214759936006 ) ) ;
#83910=CARTESIAN_POINT ( 'NONE',  ( -97.34389577676000727, -291.9992585872445829, -222.3622082161248272 ) ) ;
#83911=CARTESIAN_POINT ( 'NONE',  ( -81.89984964257409672, -291.9550836814762533, -207.6387279219162565 ) ) ;
#83912=CARTESIAN_POINT ( 'NONE',  ( 33.08247196139245716, -287.9749944389534448, -289.7694381909022923 ) ) ;
#83913=ORIENTED_EDGE ( 'NONE', *, *, #33928, .F. ) ;
#83915=CARTESIAN_POINT ( 'NONE',  ( -111.3982826323108952, -298.6166201562301126, -254.3027215100758269 ) ) ;
#83916=CARTESIAN_POINT ( 'NONE',  ( -37.58915063716619898, -296.7339469850733735, -193.8546669906522197 ) ) ;
#83918=CARTESIAN_POINT ( 'NONE',  ( 21.52523181331077851, -280.0017832391246770, -226.7729005884143305 ) ) ;
#83920=CARTESIAN_POINT ( 'NONE',  ( 36.00207379519542172, -275.3521770434582550, -293.6037023895218567 ) ) ;
#83921=CARTESIAN_POINT ( 'NONE',  ( -109.1482974707535618, -295.2485416031366299, -253.7924628518241548 ) ) ;
#83922=CARTESIAN_POINT ( 'NONE',  ( -40.53559120196599252, -278.9531250518029992, -344.5402585330048737 ) ) ;
#83923=CARTESIAN_POINT ( 'NONE',  ( 36.93432641576955433, -273.7081801739291222, -271.6293174504942272 ) ) ;
#83924=CARTESIAN_POINT ( 'NONE',  ( -101.8087998733637960, -297.2808868785924119, -305.4484882776049517 ) ) ;
#83925=CARTESIAN_POINT ( 'NONE',  ( -93.86065634821555648, -298.2910649818296633, -223.6528966957968407 ) ) ;
#83927=CARTESIAN_POINT ( 'NONE',  ( -112.8569653684336913, -298.0185950843005003, -280.9392090985708137 ) ) ;
#83928=CARTESIAN_POINT ( 'NONE',  ( -45.89534905715190405, -295.9437612415042622, -195.6827173879338204 ) ) ;
#83929=CARTESIAN_POINT ( 'NONE',  ( -70.27405572185325866, -292.2575675818152376, -205.0974020021615161 ) ) ;
#83930=CARTESIAN_POINT ( 'NONE',  ( -109.2423010203707747, -288.9210545243886372, -286.0939006829962636 ) ) ;
#83932=CARTESIAN_POINT ( 'NONE',  ( 39.56220613950321052, -276.0904791904014246, -274.0347681874903287 ) ) ;
#83933=CARTESIAN_POINT ( 'NONE',  ( -36.48735443589124117, -298.3964193980501705, -197.3399237719114012 ) ) ;
#83934=CARTESIAN_POINT ( 'NONE',  ( 29.25610738932950383, -283.0655085084358689, -234.9917681661301856 ) ) ;
#83935=CARTESIAN_POINT ( 'NONE',  ( 13.34148142253305203, -281.0456735419071492, -327.7422955045147432 ) ) ;
#83936=CARTESIAN_POINT ( 'NONE',  ( -6.623050125827185219, -276.0078979036036344, -340.8712928156508042 ) ) ;
#83937=CARTESIAN_POINT ( 'NONE',  ( -84.97463679934691072, -282.9266292620180820, -325.8922360203860080 ) ) ;
#83938=CARTESIAN_POINT ( 'NONE',  ( -11.36021665909794187, -280.7144261539231138, -340.9500234533661569 ) ) ;
#83940=CARTESIAN_POINT ( 'NONE',  ( -90.61070835319829087, -271.8534170688649851, -219.5707689357697916 ) ) ;
#83941=CARTESIAN_POINT ( 'NONE',  ( -98.82319815346400560, -281.1355286006927372, -227.3852875761047869 ) ) ;
#83944=CARTESIAN_POINT ( 'NONE',  ( -26.36916475778452096, -296.4275949629883371, -194.3776795965844144 ) ) ;
#83946=CARTESIAN_POINT ( 'NONE',  ( -70.73298100031612989, -279.4917056420243853, -337.7039037324613560 ) ) ;
#83947=CARTESIAN_POINT ( 'NONE',  ( -31.14988150182231408, -272.1301938691457849, -195.6041451806287057 ) ) ;
#83949=CARTESIAN_POINT ( 'NONE',  ( -96.46914734857280393, -287.1141152049804077, -223.3158292909071179 ) ) ;
#83952=CARTESIAN_POINT ( 'NONE',  ( -36.71322620156909977, -287.0441561253251166, -345.3710874019907919 ) ) ;
#83954=DIRECTION ( 'NONE',  ( 0.000000000000000000, 1.000000000000000000, 8.326672684688666165E-15 ) ) ;
#83955=CARTESIAN_POINT ( 'NONE',  ( 16.43970375136555973, -293.0611164902616679, -320.3080007865403900 ) ) ;
#83956=CARTESIAN_POINT ( 'NONE',  ( 31.62406566559199206, -286.0548058008955081, -297.9694226751135488 ) ) ;
#83958=CARTESIAN_POINT ( 'NONE',  ( -111.7162405794117745, -294.6811226260463741, -260.3039712180333254 ) ) ;
#83959=CARTESIAN_POINT ( 'NONE',  ( 4.812928341383445385, -285.0898429945812609, -206.6923949498348350 ) ) ;
#83960=CARTESIAN_POINT ( 'NONE',  ( 35.82316986095185740, -283.0212704428925576, -260.3205806844256358 ) ) ;
#83961=CARTESIAN_POINT ( 'NONE',  ( 21.20447964399378193, -279.1322222369270776, -221.9223024430743578 ) ) ;
#83962=CARTESIAN_POINT ( 'NONE',  ( 14.08338210787727718, -288.3050594054060412, -322.1729015556517197 ) ) ;
#83963=CARTESIAN_POINT ( 'NONE',  ( -109.1859444515794735, -280.1865814893170068, -254.3729092287918547 ) ) ;
#83964=CARTESIAN_POINT ( 'NONE',  ( -79.15551110448454608, -280.2745213306582173, -210.3260704004291881 ) ) ;
#83966=CARTESIAN_POINT ( 'NONE',  ( 34.38994614782031078, -289.8286923270100601, -293.4474283241677313 ) ) ;
#83968=CARTESIAN_POINT ( 'NONE',  ( -102.7190386961535324, -273.0843339309972180, -229.6818406812649016 ) ) ;
#83969=CARTESIAN_POINT ( 'NONE',  ( -93.63593261125106437, -291.8478009163669640, -319.4567551299195429 ) ) ;
#83971=CARTESIAN_POINT ( 'NONE',  ( -119.3990491898856732, -293.0519495502701943, -270.3937649182068412 ) ) ;
#83973=CARTESIAN_POINT ( 'NONE',  ( 37.49466387646914001, -273.4550046218384978, -262.7909252614521733 ) ) ;
#83975=CARTESIAN_POINT ( 'NONE',  ( -111.1983495673783580, -294.7143219310675022, -289.1658044707526756 ) ) ;
#83976=CARTESIAN_POINT ( 'NONE',  ( -63.09529223877257920, -297.2152696214330945, -201.9355183477014748 ) ) ;
#83977=CARTESIAN_POINT ( 'NONE',  ( -34.53236061960532055, -290.5364766707357944, -344.0509371547043997 ) ) ;
#83978=CARTESIAN_POINT ( 'NONE',  ( -70.65117173693242592, -285.2577022609833648, -336.4695633156177337 ) ) ;
#83979=CARTESIAN_POINT ( 'NONE',  ( -113.6618864241788600, -291.9305455041455843, -274.0807221493817565 ) ) ;
#83980=CARTESIAN_POINT ( 'NONE',  ( -113.5175090885641112, -291.9637155526046399, -262.7030824782200398 ) ) ;
#83981=CARTESIAN_POINT ( 'NONE',  ( -89.09244599986395485, -287.3245327898364962, -216.0761205283811250 ) ) ;
#83982=CARTESIAN_POINT ( 'NONE',  ( 17.22161360000555419, -280.9709689961040340, -215.9554727689570655 ) ) ;
#83983=CARTESIAN_POINT ( 'NONE',  ( -112.8691641132310224, -294.6776532690637964, -266.7787020702002678 ) ) ;
#83984=CARTESIAN_POINT ( 'NONE',  ( -58.48878688903942447, -283.1514003894635607, -344.4558005426727050 ) ) ;
#83985=CARTESIAN_POINT ( 'NONE',  ( 18.19411868959419820, -276.7196362612757525, -221.0240580767523966 ) ) ;
#83987=CARTESIAN_POINT ( 'NONE',  ( 30.91033621190086578, -278.2662352645559167, -285.9065529553535612 ) ) ;
#83988=CARTESIAN_POINT ( 'NONE',  ( -112.5432924226630433, -276.5692437914692050, -279.9984958808888678 ) ) ;
#83990=CARTESIAN_POINT ( 'NONE',  ( 33.82175347843743651, -280.8417223679282984, -253.8156862059487935 ) ) ;
#83991=CARTESIAN_POINT ( 'NONE',  ( -73.89380412828245426, -278.7315646660425159, -337.6958184713817559 ) ) ;
#83992=CARTESIAN_POINT ( 'NONE',  ( -102.3129323252662033, -284.1479342094740446, -229.4764118025549919 ) ) ;
#83993=CARTESIAN_POINT ( 'NONE',  ( -47.15064450055134415, -293.6859847864207609, -197.0006475479784740 ) ) ;
#83994=CARTESIAN_POINT ( 'NONE',  ( 38.12899637370343697, -277.0193627192431904, -259.8437806426530301 ) ) ;
#83995=CARTESIAN_POINT ( 'NONE',  ( 29.50842678219011717, -276.3806609960516312, -233.0452490753298207 ) ) ;
#83996=CARTESIAN_POINT ( 'NONE',  ( 34.16413500685495563, -275.5793107147000569, -285.0551829812654319 ) ) ;
#83997=CARTESIAN_POINT ( 'NONE',  ( -112.2181338329300075, -298.5374536157656848, -271.5162124592046666 ) ) ;
#83998=CARTESIAN_POINT ( 'NONE',  ( -103.8565817352469338, -283.0067381587821274, -236.0711931027333890 ) ) ;
#83999=CARTESIAN_POINT ( 'NONE',  ( 37.40243315089014686, -292.9884597069143979, -251.9475677542298797 ) ) ;
#84000=CARTESIAN_POINT ( 'NONE',  ( 22.67015429275699390, -289.7866894424861925, -317.3397510307340212 ) ) ;
#84001=CARTESIAN_POINT ( 'NONE',  ( -5.896624094609218325, -291.3958596477193055, -204.1246723523908599 ) ) ;
#84003=CARTESIAN_POINT ( 'NONE',  ( 23.51702325323197584, -291.5062184797483269, -224.1354455755057700 ) ) ;
#84004=CARTESIAN_POINT ( 'NONE',  ( -49.68812433923433503, -291.5571938979070978, -198.3399696207638101 ) ) ;
#84006=CARTESIAN_POINT ( 'NONE',  ( 18.42950154959243747, -289.3535682296907225, -323.0020295734032061 ) ) ;
#84007=CARTESIAN_POINT ( 'NONE',  ( -106.4661191018257256, -279.1999631636301160, -246.6706879880795213 ) ) ;
#84008=CARTESIAN_POINT ( 'NONE',  ( -96.28270994678318573, -294.8096868399968002, -319.4473130860597507 ) ) ;
#84009=CARTESIAN_POINT ( 'NONE',  ( -106.5909216263464288, -285.6331027402039808, -236.9267328655530775 ) ) ;
#84010=CARTESIAN_POINT ( 'NONE',  ( 25.52538447817422806, -287.2971360857175114, -225.9145936532280246 ) ) ;
#84011=CARTESIAN_POINT ( 'NONE',  ( -51.01769718933186937, -283.5649108888696333, -342.1417447864898804 ) ) ;
#84012=CARTESIAN_POINT ( 'NONE',  ( 197.4015392562739919, 285.3449900594512201, -111.8235324931284254 ) ) ;
#84013=CARTESIAN_POINT ( 'NONE',  ( -14.12022291970766474, -91.10070253271963736, -358.9863105665188527 ) ) ;
#84014=CARTESIAN_POINT ( 'NONE',  ( 200.1442466446337107, 290.5774034492648070, -82.37037781961689120 ) ) ;
#84015=CARTESIAN_POINT ( 'NONE',  ( 22.41862610576340842, -274.1612628046216855, -228.1339166947878994 ) ) ;
#84016=CARTESIAN_POINT ( 'NONE',  ( -36.47626270937693960, -275.9614166408631490, -343.6776428654442839 ) ) ;
#84017=CARTESIAN_POINT ( 'NONE',  ( -98.18144993516297347, -296.6892882913668359, -223.2436612865940333 ) ) ;
#84018=CARTESIAN_POINT ( 'NONE',  ( 200.2293796500898964, 285.8280805895519165, -96.52018796492004071 ) ) ;
#84019=CARTESIAN_POINT ( 'NONE',  ( 10.20638625574125413, -275.0971162200386857, -330.3660370820721823 ) ) ;
#84020=CARTESIAN_POINT ( 'NONE',  ( -111.2016524872315983, -274.3838737416103299, -264.8601563123276605 ) ) ;
#84022=CARTESIAN_POINT ( 'NONE',  ( -37.26588926761523624, -298.9943281909984876, -193.5956370025235458 ) ) ;
#84024=CARTESIAN_POINT ( 'NONE',  ( 30.01607260997943527, -287.6635068806872368, -241.9296167611089743 ) ) ;
#84025=CARTESIAN_POINT ( 'NONE',  ( -113.4432621766780898, -297.4892296934866636, -259.6493024644798311 ) ) ;
#84027=CARTESIAN_POINT ( 'NONE',  ( -114.0599855068598742, -297.1255947322163706, -263.8818863677628883 ) ) ;
#84028=CARTESIAN_POINT ( 'NONE',  ( 22.93419184013481882, -294.2928963507961839, -311.6298146364451895 ) ) ;
#84030=CARTESIAN_POINT ( 'NONE',  ( 36.22714454532792416, -277.2520323464382841, -253.0729878987292238 ) ) ;
#84031=CARTESIAN_POINT ( 'NONE',  ( 8.514892865990800530, -280.1687684535842209, -208.5154433925807780 ) ) ;
#84032=CARTESIAN_POINT ( 'NONE',  ( -71.75417894124989004, -278.4599248798336930, -335.0219151365827770 ) ) ;
#84033=CARTESIAN_POINT ( 'NONE',  ( 38.13383452523406447, -277.4294042609818689, -279.6021182810642927 ) ) ;
#84034=CARTESIAN_POINT ( 'NONE',  ( -68.36183585955943443, -275.4777002534902408, -339.0495065716492604 ) ) ;
#84035=CARTESIAN_POINT ( 'NONE',  ( -36.49022645758874717, -298.7145030422807395, -197.2590868350004314 ) ) ;
#84036=CARTESIAN_POINT ( 'NONE',  ( -86.90007640237055853, -294.3329166013045324, -324.7609549023745217 ) ) ;
#84038=CARTESIAN_POINT ( 'NONE',  ( 37.61612031612828133, -281.8267443075811798, -252.9581671542618437 ) ) ;
#84039=CARTESIAN_POINT ( 'NONE',  ( -109.4917394183918731, -278.5723094211032844, -281.4684054514589775 ) ) ;
#84040=CARTESIAN_POINT ( 'NONE',  ( 27.02080290780034488, -286.7842160521863661, -311.8201808807108364 ) ) ;
#84041=CARTESIAN_POINT ( 'NONE',  ( -21.03319204225030958, -300.2560068086375509, -195.1888979627098308 ) ) ;
#84043=CARTESIAN_POINT ( 'NONE',  ( -37.27811971085482412, -288.2485018991895913, -343.5225674290333018 ) ) ;
#84044=CARTESIAN_POINT ( 'NONE',  ( -32.87983607865182734, -278.3489949400248520, -196.4823944983590138 ) ) ;
#84045=CARTESIAN_POINT ( 'NONE',  ( -22.05442270774257096, -278.8264288725645201, -198.3249938738417768 ) ) ;
#84046=CARTESIAN_POINT ( 'NONE',  ( -96.27110465456443933, -282.0038381080028103, -315.8642323000574947 ) ) ;
#84047=CARTESIAN_POINT ( 'NONE',  ( -97.94282031743513528, -287.1546922776474844, -226.1525944406728286 ) ) ;
#84048=CARTESIAN_POINT ( 'NONE',  ( -99.50325845363026644, -279.2200745085292510, -309.4825682434608325 ) ) ;
#84050=CARTESIAN_POINT ( 'NONE',  ( 19.77046764803288070, -294.8791675434364947, -221.7287412414027017 ) ) ;
#84051=CARTESIAN_POINT ( 'NONE',  ( 24.07452561535351876, -276.7527802741784058, -310.1021667802164643 ) ) ;
#84052=CARTESIAN_POINT ( 'NONE',  ( -87.08866284598654772, -285.7427942203126463, -326.7801127295439869 ) ) ;
#84054=CARTESIAN_POINT ( 'NONE',  ( -112.7522582662717667, -292.5328441232037449, -265.6111793545458113 ) ) ;
#84055=CARTESIAN_POINT ( 'NONE',  ( -96.78370317882382778, -293.9252633432229231, -316.1163539989306628 ) ) ;
#84056=CARTESIAN_POINT ( 'NONE',  ( 32.56936838143245438, -286.3394379635957421, -238.3488094514989939 ) ) ;
#84057=DIRECTION ( 'NONE',  ( -1.000000000000000000, -0.000000000000000000, -0.000000000000000000 ) ) ;
#84058=CARTESIAN_POINT ( 'NONE',  ( 33.33890541901754290, -273.9703632588102664, -250.0422061126269568 ) ) ;
#84059=CARTESIAN_POINT ( 'NONE',  ( 21.48781892466489296, -292.3186021792932365, -315.6583313237310904 ) ) ;
#84061=CARTESIAN_POINT ( 'NONE',  ( -105.3770830688679041, -289.4822640335980850, -235.6918926359713566 ) ) ;
#84062=CARTESIAN_POINT ( 'NONE',  ( -109.9840649319341139, -286.3231102046467527, -257.2696543365985349 ) ) ;
#84063=CARTESIAN_POINT ( 'NONE',  ( 38.68820804717498874, -285.8071789043202671, -271.5579962621189907 ) ) ;
#84064=CARTESIAN_POINT ( 'NONE',  ( -109.2444953758464550, -286.1831778277103240, -254.6381563084175070 ) ) ;
#84066=CARTESIAN_POINT ( 'NONE',  ( -57.44855760783973864, -286.5888707866337768, -199.9641180728100949 ) ) ;
#84067=CARTESIAN_POINT ( 'NONE',  ( 3.234173688355151288, -294.5738760214815102, -206.8012072149851406 ) ) ;
#84068=CARTESIAN_POINT ( 'NONE',  ( 34.37118292351006232, -273.3247653061418987, -246.3931547603452827 ) ) ;
#84069=CARTESIAN_POINT ( 'NONE',  ( -4.000165905497466312, -276.9576899198232809, -339.7592308261783955 ) ) ;
#84070=CARTESIAN_POINT ( 'NONE',  ( 14.46890927587927855, -290.8534963126913340, -215.2894829904719529 ) ) ;
#84071=CARTESIAN_POINT ( 'NONE',  ( -96.81743442926509147, -279.2092680636500290, -221.4362485684084163 ) ) ;
#84072=CARTESIAN_POINT ( 'NONE',  ( -56.19492730656106971, -297.2759710845810446, -342.6393439620219965 ) ) ;
#84075=CARTESIAN_POINT ( 'NONE',  ( -57.51377248618479143, -284.4712050929588827, -199.6375725737202345 ) ) ;
#84076=CARTESIAN_POINT ( 'NONE',  ( -87.95470032532377047, -275.9086753290813476, -324.6675604123684025 ) ) ;
#84077=CARTESIAN_POINT ( 'NONE',  ( 29.28837393571043535, -280.0076609207429783, -304.7912483337048570 ) ) ;
#84079=CARTESIAN_POINT ( 'NONE',  ( 0.8651884253017493309, -273.0320172676609900, -204.2934029561769478 ) ) ;
#84080=CARTESIAN_POINT ( 'NONE',  ( -89.16392737490745901, -277.1532573706602989, -321.9921915233116465 ) ) ;
#84082=CARTESIAN_POINT ( 'NONE',  ( -20.67270286735145390, -296.3545195133043535, -342.1970915529847730 ) ) ;
#84083=CARTESIAN_POINT ( 'NONE',  ( -14.30744618961798587, -279.2642055532322161, -197.1554856837258853 ) ) ;
#84084=CARTESIAN_POINT ( 'NONE',  ( -23.46253366839147247, -295.8117527629580650, -342.3210061666968613 ) ) ;
#84085=CARTESIAN_POINT ( 'NONE',  ( -113.8450012276363452, -297.8766016269611896, -269.6241021796294035 ) ) ;
#84086=CARTESIAN_POINT ( 'NONE',  ( -107.9594333187077666, -272.4664596222390287, -251.5870827923643560 ) ) ;
#84087=CARTESIAN_POINT ( 'NONE',  ( -73.61600686124847925, -293.5712964401704994, -204.6584400530958874 ) ) ;
#84088=CARTESIAN_POINT ( 'NONE',  ( -60.51194358135362705, -285.9265441287558360, -196.8743503303824411 ) ) ;
#84089=CARTESIAN_POINT ( 'NONE',  ( 25.03623571854281593, -274.2698057247270071, -313.4553565712622003 ) ) ;
#84090=CARTESIAN_POINT ( 'NONE',  ( -70.64099185393729385, -289.3124471222094485, -339.8029557224502923 ) ) ;
#84091=CARTESIAN_POINT ( 'NONE',  ( -111.2540434131667837, -280.6712590650361108, -259.5703077420575937 ) ) ;
#84093=CARTESIAN_POINT ( 'NONE',  ( 33.30570359326348751, -286.8672414200647154, -289.8456332267057292 ) ) ;
#84094=CARTESIAN_POINT ( 'NONE',  ( -97.58256009286091626, -289.1620496524165560, -225.6625560703271560 ) ) ;
#84096=CARTESIAN_POINT ( 'NONE',  ( 176.3450237082407170, 252.7779579681928510, -162.7338909149122799 ) ) ;
#84097=CARTESIAN_POINT ( 'NONE',  ( 16.05165294194905101, -287.7771754688169494, -320.3063537571177903 ) ) ;
#84099=CARTESIAN_POINT ( 'NONE',  ( 1.983925090223331411, -283.4804891399954272, -336.2877090822796049 ) ) ;
#84100=CARTESIAN_POINT ( 'NONE',  ( -50.51415945297529930, -290.9466217737974034, -194.7350211132831532 ) ) ;
#84101=CARTESIAN_POINT ( 'NONE',  ( -14.48732101090178581, -281.9435737816559708, -197.6138661300338413 ) ) ;
#84102=CARTESIAN_POINT ( 'NONE',  ( 35.69988107971254720, -282.5794911401022773, -247.5965471005750373 ) ) ;
#84103=CARTESIAN_POINT ( 'NONE',  ( 22.11472592452164676, -280.7938085092188203, -228.0062669549850227 ) ) ;
#84104=CARTESIAN_POINT ( 'NONE',  ( -32.58905962465235717, -276.1122001142012437, -195.4989794687439826 ) ) ;
#84105=CARTESIAN_POINT ( 'NONE',  ( 15.47868649755001336, -294.3296984442216626, -326.3879575928647796 ) ) ;
#84106=CARTESIAN_POINT ( 'NONE',  ( -101.1038103990866261, -289.0950241070623292, -231.5508088503772797 ) ) ;
#84107=CARTESIAN_POINT ( 'NONE',  ( -93.20608206901290771, -272.0207578132187791, -222.7360364352874740 ) ) ;
#84109=CARTESIAN_POINT ( 'NONE',  ( -110.8468703588214197, -286.6254919794216107, -258.5199343540625136 ) ) ;
#84110=CARTESIAN_POINT ( 'NONE',  ( 36.80126305851634783, -294.8782301631092082, -289.9650339302096427 ) ) ;
#84111=CARTESIAN_POINT ( 'NONE',  ( 15.90579520830188009, -282.9242760943060944, -320.5200533919816053 ) ) ;
#84112=CARTESIAN_POINT ( 'NONE',  ( -37.13965649441264105, -276.1083988886247766, -347.1385774689009054 ) ) ;
#84113=CARTESIAN_POINT ( 'NONE',  ( -99.95288238541117209, -291.7956531773915003, -225.7163798482874029 ) ) ;
#84114=CARTESIAN_POINT ( 'NONE',  ( -111.1509623143276002, -282.9091233968073311, -253.2585362915878875 ) ) ;
#84115=CARTESIAN_POINT ( 'NONE',  ( -16.63638181658769710, -292.6458551365373069, -196.2191320025335983 ) ) ;
#84116=CARTESIAN_POINT ( 'NONE',  ( -80.41655661549687295, -289.9870829716154503, -329.3871107777642351 ) ) ;
#84119=CARTESIAN_POINT ( 'NONE',  ( -62.54974233798310479, -182.8716734317700059, -358.6490213108781973 ) ) ;
#84120=CARTESIAN_POINT ( 'NONE',  ( -4.445045077233600317, -284.1466242025010160, -339.2268973405530801 ) ) ;
#84121=CARTESIAN_POINT ( 'NONE',  ( 31.98288692825983404, -278.6237833571634610, -237.0123917617631264 ) ) ;
#84123=CARTESIAN_POINT ( 'NONE',  ( 33.25342124041803515, -280.7325826534128623, -290.1235802061776781 ) ) ;
#84124=CARTESIAN_POINT ( 'NONE',  ( 20.80149208380332126, -275.9009877011904450, -320.8301847100901796 ) ) ;
#84125=CARTESIAN_POINT ( 'NONE',  ( -62.95991740281284166, -281.7181222957968885, -199.9947108669112197 ) ) ;
#84126=CARTESIAN_POINT ( 'NONE',  ( -92.74527687321815961, -240.5677590599414657, -340.2624655071006146 ) ) ;
#84127=CARTESIAN_POINT ( 'NONE',  ( -7.748305180309949414, -279.0071776040894065, -199.8995148093826231 ) ) ;
#84128=CARTESIAN_POINT ( 'NONE',  ( -108.5626032521937390, -282.2825884632986799, -292.7090431918928743 ) ) ;
#84129=CARTESIAN_POINT ( 'NONE',  ( -54.38989971596161155, -299.5961930513086600, -196.3115879226694744 ) ) ;
#84130=CARTESIAN_POINT ( 'NONE',  ( 20.57582070407850239, -294.6709846207678538, -314.9186583508529793 ) ) ;
#84132=CARTESIAN_POINT ( 'NONE',  ( -110.8000162012403393, -289.1903879318553550, -273.9162240245674980 ) ) ;
#84133=CARTESIAN_POINT ( 'NONE',  ( 12.64465708859684057, -277.0275570290629048, -328.7963545995968389 ) ) ;
#84134=CARTESIAN_POINT ( 'NONE',  ( -11.49022063468854782, -274.3983538089536864, -202.0377449000611989 ) ) ;
#84135=CARTESIAN_POINT ( 'NONE',  ( -32.68756867312436043, -273.0298186576122816, -193.7984835137264952 ) ) ;
#84137=CARTESIAN_POINT ( 'NONE',  ( 26.19300043881516160, -273.0152211563179776, -230.4115952906718690 ) ) ;
#84140=CARTESIAN_POINT ( 'NONE',  ( 27.13341569566594202, -283.1058317379639107, -305.2493038379324730 ) ) ;
#84141=CARTESIAN_POINT ( 'NONE',  ( 38.69629718477778368, -283.3066217929751360, -269.9135659252942219 ) ) ;
#84142=CARTESIAN_POINT ( 'NONE',  ( -91.74644881309394862, -283.2027375975015389, -319.2063423743621229 ) ) ;
#84143=CARTESIAN_POINT ( 'NONE',  ( 34.66943698811905250, -274.1635129507852184, -286.5689475532380470 ) ) ;
#84144=CARTESIAN_POINT ( 'NONE',  ( 20.62593492646530535, -282.7682556194789640, -223.9863536133989896 ) ) ;
#84145=CARTESIAN_POINT ( 'NONE',  ( 34.80405991124247578, -273.8349051508639604, -255.2762199965054037 ) ) ;
#84147=CARTESIAN_POINT ( 'NONE',  ( 31.40343704952015003, -276.2937203482857171, -244.8987499155447836 ) ) ;
#84150=CARTESIAN_POINT ( 'NONE',  ( -98.45415997985492140, -279.9774089783627460, -223.7625830552324544 ) ) ;
#84153=CARTESIAN_POINT ( 'NONE',  ( -82.55801139516458420, -287.3026708528473705, -209.5026648110881240 ) ) ;
#84154=CARTESIAN_POINT ( 'NONE',  ( -92.31875823276899951, -295.0617875245883965, -318.6324843339914992 ) ) ;
#84155=CARTESIAN_POINT ( 'NONE',  ( -73.13379150882238378, -288.8625063329561726, -338.4364093612530269 ) ) ;
#84156=CARTESIAN_POINT ( 'NONE',  ( 35.96089839981687675, -285.9263390169773515, -280.6856460144163066 ) ) ;
#84157=CARTESIAN_POINT ( 'NONE',  ( 36.14220381956344141, -286.0641268539903308, -265.5662513061336085 ) ) ;
#84158=CARTESIAN_POINT ( 'NONE',  ( -70.65704831901292948, -289.8464033489443636, -204.2698054596178565 ) ) ;
#84159=CARTESIAN_POINT ( 'NONE',  ( -110.7876435044199894, -285.7498025887919653, -270.9275964226225142 ) ) ;
#84160=CARTESIAN_POINT ( 'NONE',  ( 28.76779551838724203, -274.0232732276390379, -305.8901265657968338 ) ) ;
#84161=CARTESIAN_POINT ( 'NONE',  ( 25.70701391029787430, -285.3816485845841271, -227.5441083139265004 ) ) ;
#84162=CARTESIAN_POINT ( 'NONE',  ( -74.80360609122205062, -299.5540184186752413, -205.3276152594367829 ) ) ;
#84163=CARTESIAN_POINT ( 'NONE',  ( 36.02969781357911927, -285.7619569170653904, -286.7497145249767527 ) ) ;
#84164=CARTESIAN_POINT ( 'NONE',  ( 26.65866895623448229, -282.0082202143072436, -234.7611010640310383 ) ) ;
#84165=CARTESIAN_POINT ( 'NONE',  ( 9.115335023604126619, -290.4166657407828893, -329.5185726309060783 ) ) ;
#84168=CARTESIAN_POINT ( 'NONE',  ( -16.87301355762895838, -296.7101221609414097, -343.1500955663910872 ) ) ;
#84169=CARTESIAN_POINT ( 'NONE',  ( -62.96904363096327018, -277.7184462703167469, -199.8205644995465775 ) ) ;
#84170=CARTESIAN_POINT ( 'NONE',  ( -7.244010252994506516, -291.6341529826215151, -199.6482547733304216 ) ) ;
#84171=CARTESIAN_POINT ( 'NONE',  ( -108.6028786984695245, -295.2033262722978293, -251.1217236364072107 ) ) ;
#84172=CARTESIAN_POINT ( 'NONE',  ( 36.18112764911198553, -280.2137410495790846, -268.5882797660400456 ) ) ;
#84173=CARTESIAN_POINT ( 'NONE',  ( -5.898930076963702973, -272.5486131059699346, -202.8876682933949098 ) ) ;
#84174=CARTESIAN_POINT ( 'NONE',  ( 8.549077850769588593, -295.7238615259028620, -327.8310636730936949 ) ) ;
#84175=CARTESIAN_POINT ( 'NONE',  ( -85.28047601435906699, -292.1948066931273615, -330.5268031993605859 ) ) ;
#84176=CARTESIAN_POINT ( 'NONE',  ( -100.1687146882973707, -295.6092577201411586, -227.0314204285537016 ) ) ;
#84177=CARTESIAN_POINT ( 'NONE',  ( 28.68293991188527770, -292.2882148593819807, -308.0801322233219253 ) ) ;
#84178=CARTESIAN_POINT ( 'NONE',  ( -92.84427723113695663, -291.2932706284533992, -318.7574151495228989 ) ) ;
#84180=CARTESIAN_POINT ( 'NONE',  ( -93.57048950920508901, -292.0177802440592814, -223.5342393360562880 ) ) ;
#84182=CARTESIAN_POINT ( 'NONE',  ( -97.83654019666998636, -291.1263561124667376, -317.3545541766117708 ) ) ;
#84183=CARTESIAN_POINT ( 'NONE',  ( 8.194400807653430263, -280.4528263285691878, -330.4016901932679389 ) ) ;
#84184=CARTESIAN_POINT ( 'NONE',  ( 4.503643228094607487, -292.6340986130241504, -210.4830406153735964 ) ) ;
#84185=CARTESIAN_POINT ( 'NONE',  ( -1.135436626899125612, -280.5191310572261614, -202.4044664811583516 ) ) ;
#84186=CARTESIAN_POINT ( 'NONE',  ( -55.70125157486767620, -282.9489716560196939, -345.1185334148008792 ) ) ;
#84187=CARTESIAN_POINT ( 'NONE',  ( 22.62777516957125812, -286.1649596509760727, -315.1451604383891549 ) ) ;
#84188=CARTESIAN_POINT ( 'NONE',  ( -87.78525365492930632, -281.9051142254384104, -324.8953381684161741 ) ) ;
#84189=CARTESIAN_POINT ( 'NONE',  ( 35.51949101257611829, -279.7446526922947214, -247.6905516401435818 ) ) ;
#84190=CARTESIAN_POINT ( 'NONE',  ( 1.377537695269205109, -285.4770654264762584, -204.1467979895461156 ) ) ;
#84192=CARTESIAN_POINT ( 'NONE',  ( 9.339282516053144079, -294.3057976799779567, -213.1343177603512800 ) ) ;
#84193=CARTESIAN_POINT ( 'NONE',  ( -20.24018534709207273, -278.2620162812407330, -344.8878623916620541 ) ) ;
#84194=CARTESIAN_POINT ( 'NONE',  ( -53.96286600050149929, -276.9380423148875252, -341.5175946211983842 ) ) ;
#84196=CARTESIAN_POINT ( 'NONE',  ( -108.3679536379200101, -291.0970613800869842, -240.6244181514893796 ) ) ;
#84197=CARTESIAN_POINT ( 'NONE',  ( 14.74289963233940881, -280.4051358223019861, -325.1014930634581219 ) ) ;
#84198=CARTESIAN_POINT ( 'NONE',  ( 34.55308431079621556, -292.7943042307796873, -284.3091794673383106 ) ) ;
#84199=CARTESIAN_POINT ( 'NONE',  ( -81.76492123804200673, -295.4474594584571605, -209.8683182010375106 ) ) ;
#84202=CARTESIAN_POINT ( 'NONE',  ( 31.59603316035471821, -293.3832952224719293, -294.7112702006300538 ) ) ;
#84204=CARTESIAN_POINT ( 'NONE',  ( 7.450504543161054372, -290.1952119285918457, -214.2458315076590907 ) ) ;
#84205=CARTESIAN_POINT ( 'NONE',  ( -113.7010580509932538, -271.8566991735337410, -261.7933132546746151 ) ) ;
#84206=CARTESIAN_POINT ( 'NONE',  ( 29.96875611653377547, -280.1473829829694751, -305.1405365804114354 ) ) ;
#84207=CARTESIAN_POINT ( 'NONE',  ( 32.25640295642875088, -288.4571037273194634, -238.4625537657218786 ) ) ;
#84208=CARTESIAN_POINT ( 'NONE',  ( -10.74799410011047129, -286.2421762419389779, -202.3639556289292898 ) ) ;
#84209=CARTESIAN_POINT ( 'NONE',  ( -64.57149029116656891, -278.9341917377763025, -338.8933746296383447 ) ) ;
#84210=CARTESIAN_POINT ( 'NONE',  ( -93.44316806302283851, -293.8849180890236426, -319.6000466888648930 ) ) ;
#84211=CARTESIAN_POINT ( 'NONE',  ( -82.96710108700392539, -297.4459863385596918, -328.7042018548107194 ) ) ;
#84212=CARTESIAN_POINT ( 'NONE',  ( -104.6415815996227821, -276.9538819635504296, -299.7777200734809071 ) ) ;
#84214=CARTESIAN_POINT ( 'NONE',  ( -93.67689133787453670, -295.5033907039386349, -322.8409040926529769 ) ) ;
#84215=CARTESIAN_POINT ( 'NONE',  ( -111.6853062565581354, -292.5330151408027746, -265.6687439620454256 ) ) ;
#84216=CARTESIAN_POINT ( 'NONE',  ( 24.25178145173790512, -295.7541794308115755, -315.2460453000618941 ) ) ;
#84218=CARTESIAN_POINT ( 'NONE',  ( 14.16107102299992881, -288.9563676298772634, -322.2394104740536704 ) ) ;
#84220=CARTESIAN_POINT ( 'NONE',  ( 13.51590753469923634, -281.4195353792096057, -327.9325061032266717 ) ) ;
#84221=CARTESIAN_POINT ( 'NONE',  ( -114.0198772851753972, -297.2846351305698818, -263.8873078390062119 ) ) ;
#84222=CARTESIAN_POINT ( 'NONE',  ( -99.01164022056724434, -289.2842297449119542, -226.3483474409320024 ) ) ;
#84223=CARTESIAN_POINT ( 'NONE',  ( -78.19483769674188522, -297.8518938605167818, -205.1172259904422219 ) ) ;
#84227=CARTESIAN_POINT ( 'NONE',  ( -65.17591355673499720, -290.9293396260902682, -341.4659743038619695 ) ) ;
#84228=CARTESIAN_POINT ( 'NONE',  ( -72.08107566293803359, -276.1233781216987495, -198.2974183793908196 ) ) ;
#84229=CARTESIAN_POINT ( 'NONE',  ( 38.76919227837110782, -281.0381773904672968, -281.3358545929219758 ) ) ;
#84230=CARTESIAN_POINT ( 'NONE',  ( -107.2873500578149191, -286.8987710344947004, -243.7597180105432244 ) ) ;
#84231=CARTESIAN_POINT ( 'NONE',  ( -21.09144749120965301, -284.8314473139080292, -195.6983054148370798 ) ) ;
#84232=CARTESIAN_POINT ( 'NONE',  ( 26.86152152137588800, -273.0349971875366464, -231.8162567734447350 ) ) ;
#84233=CARTESIAN_POINT ( 'NONE',  ( -34.00003006958469598, -276.0146693112488379, -195.9961568719902516 ) ) ;
#84234=CARTESIAN_POINT ( 'NONE',  ( -111.1241051553056138, -288.7646465966976734, -260.1069912797450456 ) ) ;
#84235=CARTESIAN_POINT ( 'NONE',  ( -109.4831368209674167, -280.1148041854552275, -293.6797821124986854 ) ) ;
#84237=CARTESIAN_POINT ( 'NONE',  ( -34.31332839501501297, -280.0912474586286862, -197.4114168354948049 ) ) ;
#84238=CARTESIAN_POINT ( 'NONE',  ( 35.52990753708684224, -280.9851388785493214, -276.7683184864600321 ) ) ;
#84239=CARTESIAN_POINT ( 'NONE',  ( 24.12817021593569677, -277.2442940841727932, -316.2190240676875419 ) ) ;
#84240=CARTESIAN_POINT ( 'NONE',  ( -33.91758640765102228, -278.8892612368916275, -193.8347554364740120 ) ) ;
#84241=CARTESIAN_POINT ( 'NONE',  ( -111.8926394666918753, -268.1718929385297088, -295.4674195431252315 ) ) ;
#84242=CARTESIAN_POINT ( 'NONE',  ( 23.33944059232405266, -277.1233348428481804, -317.3996648747249765 ) ) ;
#84243=CARTESIAN_POINT ( 'NONE',  ( -30.56796663164417893, -299.5606560979661026, -193.9487378532710693 ) ) ;
#84244=CARTESIAN_POINT ( 'NONE',  ( 39.58706461736021254, -284.0519495502703080, -270.3284710469133074 ) ) ;
#84247=CARTESIAN_POINT ( 'NONE',  ( 35.26844308098985437, -288.7656935109196752, -280.5518043419718310 ) ) ;
#84248=CARTESIAN_POINT ( 'NONE',  ( 29.48237270153248701, -289.7877105833223368, -306.6446534734146212 ) ) ;
#84249=CARTESIAN_POINT ( 'NONE',  ( -109.2807042682991323, -289.7296501273459626, -283.3485100116148487 ) ) ;
#84250=CARTESIAN_POINT ( 'NONE',  ( -87.70492119207074211, -284.8785635359379853, -212.1264027678606681 ) ) ;
#84251=CARTESIAN_POINT ( 'NONE',  ( -38.48138622635112682, -140.2860406175970525, -364.7253011062631458 ) ) ;
#84252=CARTESIAN_POINT ( 'NONE',  ( 35.01099711661705527, -280.1426295613439379, -284.9686179619862969 ) ) ;
#84253=CARTESIAN_POINT ( 'NONE',  ( 10.93623958309508915, -290.2367336015209389, -326.8215340460706102 ) ) ;
#84254=CARTESIAN_POINT ( 'NONE',  ( -95.67704250042621084, -282.4038054844089629, -315.4116642789221032 ) ) ;
#84256=CARTESIAN_POINT ( 'NONE',  ( -49.23812023226650325, -281.2125347697121924, -197.8372000961076935 ) ) ;
#84257=CARTESIAN_POINT ( 'NONE',  ( -61.80452772538647821, -277.8710622567538735, -339.2593536484066021 ) ) ;
#84258=CARTESIAN_POINT ( 'NONE',  ( -111.8799066240244429, -289.1243022832196061, -288.0826368843599994 ) ) ;
#84259=CARTESIAN_POINT ( 'NONE',  ( -109.1483938591909464, -285.0063924531587531, -297.8581417460736702 ) ) ;
#84260=CARTESIAN_POINT ( 'NONE',  ( -97.99203856796732737, -284.4114506142909136, -317.7009886062413671 ) ) ;
#84261=CARTESIAN_POINT ( 'NONE',  ( -7.251538131411003008, -282.8128350608000687, -336.8848472271125161 ) ) ;
#84262=ORIENTED_EDGE ( 'NONE', *, *, #7422, .T. ) ;
#84264=CARTESIAN_POINT ( 'NONE',  ( -76.55065144290706769, -293.3943204828004809, -205.4703344455697618 ) ) ;
#84265=CARTESIAN_POINT ( 'NONE',  ( -95.27644711963867508, -289.9162994454585487, -220.3724753208754805 ) ) ;
#84266=CARTESIAN_POINT ( 'NONE',  ( 23.99709799971681434, -274.0582521734554007, -230.3491161291757976 ) ) ;
#84267=CARTESIAN_POINT ( 'NONE',  ( -84.12976630326390648, -295.0246793856765066, -331.4543991745005087 ) ) ;
#84268=CARTESIAN_POINT ( 'NONE',  ( -98.86782811605233690, -289.5903964135389401, -229.7068626942543688 ) ) ;
#84269=CARTESIAN_POINT ( 'NONE',  ( -53.39064865174962193, -293.5005271629672734, -342.6661994042524952 ) ) ;
#84270=CARTESIAN_POINT ( 'NONE',  ( -109.8087082694134295, -291.6033783781911666, -282.0875244714740688 ) ) ;
#84272=CARTESIAN_POINT ( 'NONE',  ( -109.9785144731161211, -292.3117252170790721, -289.0911257362126889 ) ) ;
#84273=CARTESIAN_POINT ( 'NONE',  ( -33.60442121298309104, -290.0989374290365390, -195.2874130339217515 ) ) ;
#84274=CARTESIAN_POINT ( 'NONE',  ( -58.64995643420090232, -297.3277305333636491, -342.3238007217727841 ) ) ;
#84275=CARTESIAN_POINT ( 'NONE',  ( -10.67542976517641229, -287.3499294775880344, -202.1396432910799206 ) ) ;
#84276=CARTESIAN_POINT ( 'NONE',  ( 37.00701095535362128, -295.6939918885259999, -281.4199419344276407 ) ) ;
#84277=CARTESIAN_POINT ( 'NONE',  ( 37.50697896403737275, -277.6491198010464814, -279.5223611885564310 ) ) ;
#84278=CARTESIAN_POINT ( 'NONE',  ( -70.64977880336589067, -296.8211718963902968, -201.1171239006658595 ) ) ;
#84279=CARTESIAN_POINT ( 'NONE',  ( -35.10921939121834612, -275.2635925825913432, -344.3407776557868374 ) ) ;
#84280=CARTESIAN_POINT ( 'NONE',  ( -92.34465615442489650, -277.3374061754516333, -220.2014825459703786 ) ) ;
#84281=CARTESIAN_POINT ( 'NONE',  ( -108.9255479152700303, -273.9699580531637935, -254.1474434379779552 ) ) ;
#84282=CARTESIAN_POINT ( 'NONE',  ( 29.44144410201021955, -273.6406558548493422, -233.1225251567176144 ) ) ;
#84283=CARTESIAN_POINT ( 'NONE',  ( -99.21899739887237502, -297.4294650509331177, -310.2862679077778125 ) ) ;
#84285=CARTESIAN_POINT ( 'NONE',  ( -108.3341153041739631, -297.5884285414779242, -252.6270757957564967 ) ) ;
#84287=CARTESIAN_POINT ( 'NONE',  ( -88.39602578302967117, -287.7836040645354956, -325.7855046044128358 ) ) ;
#84288=CARTESIAN_POINT ( 'NONE',  ( -60.51589897267113116, -297.7431833686640630, -201.0836897982399591 ) ) ;
#84289=CARTESIAN_POINT ( 'NONE',  ( -30.88385360709938965, -286.1316094809763513, -193.6191048309662506 ) ) ;
#84290=CARTESIAN_POINT ( 'NONE',  ( -74.42085929146699641, -289.1980951366976456, -337.8363800987611967 ) ) ;
#84291=CARTESIAN_POINT ( 'NONE',  ( -111.7690686305628844, -298.6837421102805479, -258.4904968765356443 ) ) ;
#84292=CARTESIAN_POINT ( 'NONE',  ( 7.132559714435090292, -292.4450679489729623, -330.6093050559271092 ) ) ;
#84293=CARTESIAN_POINT ( 'NONE',  ( 26.15296653694375806, -280.1763454094890449, -226.9948738121624956 ) ) ;
#84294=CARTESIAN_POINT ( 'NONE',  ( 39.58706461736020543, -291.0523547857347353, -270.3937649182068981 ) ) ;
#84295=CARTESIAN_POINT ( 'NONE',  ( -103.3591830014524078, -276.0782298887147590, -306.0594822812865345 ) ) ;
#84297=CARTESIAN_POINT ( 'NONE',  ( -84.95421151834061391, -288.5208364814200763, -326.2867783800795110 ) ) ;
#84299=CARTESIAN_POINT ( 'NONE',  ( -20.70994004439706160, -286.8384563345694573, -343.4937728102298706 ) ) ;
#84300=CARTESIAN_POINT ( 'NONE',  ( -47.40174905920618897, -299.5224585793560550, -197.1982248599935303 ) ) ;
#84301=CARTESIAN_POINT ( 'NONE',  ( 0.5917316778180724546, -283.9821162239069849, -336.7061761888923570 ) ) ;
#84302=CARTESIAN_POINT ( 'NONE',  ( -110.4191644669191419, -270.8793731151073985, -250.9517806020308797 ) ) ;
#84303=CARTESIAN_POINT ( 'NONE',  ( 34.56709077066861369, -281.3862695652334196, -257.7863101717085215 ) ) ;
#84304=CARTESIAN_POINT ( 'NONE',  ( -66.05969493943618431, -275.0940551891459336, -202.6067698408761828 ) ) ;
#84305=CARTESIAN_POINT ( 'NONE',  ( -22.97491304383034461, -282.2359772161225351, -196.6971608211119644 ) ) ;
#84306=CARTESIAN_POINT ( 'NONE',  ( -79.01955879049030784, -272.3960262269687291, -209.9904073063051158 ) ) ;
#84308=CARTESIAN_POINT ( 'NONE',  ( 204.9104695348173095, 293.4474168480153367, -54.00000000001035971 ) ) ;
#84309=CARTESIAN_POINT ( 'NONE',  ( -110.5887428641317030, -286.3465580144860496, -284.7387928971211863 ) ) ;
#84311=CARTESIAN_POINT ( 'NONE',  ( 13.79469577742117181, -279.9094976428775681, -334.5364918783848793 ) ) ;
#84312=CARTESIAN_POINT ( 'NONE',  ( -113.6072760330506810, -277.6266566226042869, -280.1487678197534592 ) ) ;
#84313=CARTESIAN_POINT ( 'NONE',  ( -111.8533543602551674, -289.1543620381488040, -254.3480278353933954 ) ) ;
#84314=CARTESIAN_POINT ( 'NONE',  ( -45.69905321739354065, -284.6799852293620461, -343.6305057929895383 ) ) ;
#84315=CARTESIAN_POINT ( 'NONE',  ( 34.67840892800860075, -277.3632515014755882, -286.5290304503243419 ) ) ;
#84316=CARTESIAN_POINT ( 'NONE',  ( -76.44066801212321138, -284.9891923656160770, -336.0721096760068463 ) ) ;
#84317=CARTESIAN_POINT ( 'NONE',  ( -108.1482501991677196, -283.0925459854659607, -289.7363837125326995 ) ) ;
#84318=CARTESIAN_POINT ( 'NONE',  ( 26.83482368570765075, -283.0311184685040757, -231.4484905653811495 ) ) ;
#84319=CARTESIAN_POINT ( 'NONE',  ( -44.04487388210681331, -274.1364358827622709, -193.6001342238260747 ) ) ;
#84320=CARTESIAN_POINT ( 'NONE',  ( -35.71363750593609865, -276.8656109619170138, -347.3570280709755025 ) ) ;
#84322=CARTESIAN_POINT ( 'NONE',  ( -98.34979951904632856, -297.8890285824146531, -313.0146759535410865 ) ) ;
#84325=CARTESIAN_POINT ( 'NONE',  ( -113.1312661829077939, -294.6656637271667591, -272.4123263554637902 ) ) ;
#84326=CARTESIAN_POINT ( 'NONE',  ( 22.33471725297932409, -274.4716980474815955, -228.1883773466636001 ) ) ;
#84327=CARTESIAN_POINT ( 'NONE',  ( -102.3900012608572894, -274.2892154395384523, -229.9046322508898754 ) ) ;
#84328=CARTESIAN_POINT ( 'NONE',  ( -11.69152912976776015, -288.1509467107841829, -200.9345903366583457 ) ) ;
#84329=CARTESIAN_POINT ( 'NONE',  ( 38.81164438414817397, -295.1430409420499359, -275.9687372257406537 ) ) ;
#84330=CARTESIAN_POINT ( 'NONE',  ( 38.45669660543479296, -294.6135550070981708, -258.9326703334056674 ) ) ;
#84331=CARTESIAN_POINT ( 'NONE',  ( -110.2185687365378755, -292.7717898334248616, -253.3054367167377166 ) ) ;
#84332=CARTESIAN_POINT ( 'NONE',  ( -103.7719087966673328, -277.0104159909346890, -235.7947370955506585 ) ) ;
#84333=CARTESIAN_POINT ( 'NONE',  ( -111.7921871291635227, -280.5043544641291646, -267.8842725255389610 ) ) ;
#84334=CARTESIAN_POINT ( 'NONE',  ( -102.7439189514116009, -294.1561601731656879, -305.9119825044945742 ) ) ;
#84335=CARTESIAN_POINT ( 'NONE',  ( -52.64459181559339385, -285.1064613516277291, -344.6180137707083873 ) ) ;
#84336=CARTESIAN_POINT ( 'NONE',  ( -109.2293978309542268, -283.6611915346845763, -255.9950122671550901 ) ) ;
#84337=CARTESIAN_POINT ( 'NONE',  ( -61.61430774310042580, -183.8251665614383228, -361.5569093710298034 ) ) ;
#84339=CARTESIAN_POINT ( 'NONE',  ( -46.72338182567795428, -285.5966199948400117, -197.8943661436944410 ) ) ;
#84341=CARTESIAN_POINT ( 'NONE',  ( 19.56342512254201793, -283.3334309873904431, -321.8518551017077129 ) ) ;
#84342=CARTESIAN_POINT ( 'NONE',  ( -85.32725245791327495, -273.7009403575781334, -215.2530619841450630 ) ) ;
#84343=CARTESIAN_POINT ( 'NONE',  ( -46.44302071083694727, -284.7340151941835984, -194.3007821850058576 ) ) ;
#84344=CARTESIAN_POINT ( 'NONE',  ( 36.37041645891896735, -282.2232715441088544, -248.8817054813272023 ) ) ;
#84346=( NAMED_UNIT ( * ) SI_UNIT ( $, .STERADIAN. ) SOLID_ANGLE_UNIT ( ) );
#84347=CARTESIAN_POINT ( 'NONE',  ( -102.9992587898963734, -279.5599439612599326, -309.3464719749004530 ) ) ;
#84348=CARTESIAN_POINT ( 'NONE',  ( -48.11272034212307602, -280.5700980686265780, -194.1673551957038626 ) ) ;
#84349=CARTESIAN_POINT ( 'NONE',  ( -109.1418805571601069, -288.0523547857347353, -270.3284710469131937 ) ) ;
#84350=CARTESIAN_POINT ( 'NONE',  ( 139.9169389161443746, 180.0772412164195089, -241.5140256757101724 ) ) ;
#84352=CARTESIAN_POINT ( 'NONE',  ( -0.8503445863359465617, -276.5380006608442613, -205.0133822907053229 ) ) ;
#84353=CARTESIAN_POINT ( 'NONE',  ( 84.07519268682317204, 83.49645322921298884, -302.1015330633007352 ) ) ;
#84354=CARTESIAN_POINT ( 'NONE',  ( -109.1949021511918403, -276.8342382650922104, -250.0909398370305041 ) ) ;
#84355=CARTESIAN_POINT ( 'NONE',  ( 5.900922189190457523, -294.3898997889865541, -207.8787234470421765 ) ) ;
#84356=CARTESIAN_POINT ( 'NONE',  ( -101.5608122019473285, -295.4246967784312687, -305.2867291056866748 ) ) ;
#84357=CARTESIAN_POINT ( 'NONE',  ( -50.54962184610741360, -291.3954542983861984, -194.5648271302828221 ) ) ;
#84358=CARTESIAN_POINT ( 'NONE',  ( -76.79367488908245321, -294.1437925783213814, -335.8608054209029774 ) ) ;
#84359=CARTESIAN_POINT ( 'NONE',  ( 16.58171999673249886, -286.6695730069550336, -320.8214340023699265 ) ) ;
#84360=CARTESIAN_POINT ( 'NONE',  ( 36.43725941849402261, -295.5250492921121008, -279.0316752182571349 ) ) ;
#84361=CARTESIAN_POINT ( 'NONE',  ( 26.11344774377200650, -286.7436832053563762, -307.5384696529426947 ) ) ;
#84362=CARTESIAN_POINT ( 'NONE',  ( -110.3607346243348388, -285.7523831779633383, -279.1337361894713922 ) ) ;
#84364=CARTESIAN_POINT ( 'NONE',  ( -107.0518029872466030, -291.9072968687473804, -238.0891048993933623 ) ) ;
#84365=CARTESIAN_POINT ( 'NONE',  ( 15.87498493154905077, -282.7652357374507233, -320.4938084887062928 ) ) ;
#84366=CARTESIAN_POINT ( 'NONE',  ( -97.10733412382995766, -294.7015391982949950, -318.2992873502142857 ) ) ;
#84367=CARTESIAN_POINT ( 'NONE',  ( -113.6519345078848886, -291.2367556376891571, -279.7946161701090659 ) ) ;
#84368=CARTESIAN_POINT ( 'NONE',  ( -114.1268187167687813, -291.1052671532131058, -265.5059695395955828 ) ) ;
#84369=CARTESIAN_POINT ( 'NONE',  ( 29.42591672402162573, -288.1175250328088282, -300.0006963423217030 ) ) ;
#84372=CARTESIAN_POINT ( 'NONE',  ( -70.24960168051377707, -297.3414984183879710, -338.6203604525887272 ) ) ;
#84373=CARTESIAN_POINT ( 'NONE',  ( -34.05635408497725791, -296.7773065497834750, -193.8549816543329314 ) ) ;
#84375=CARTESIAN_POINT ( 'NONE',  ( 26.67029487730599868, -280.1260193048545375, -234.7820097453027870 ) ) ;
#84377=CARTESIAN_POINT ( 'NONE',  ( 23.58795260609568700, -274.4320967767723118, -223.3598426134718977 ) ) ;
#84378=CARTESIAN_POINT ( 'NONE',  ( -55.44543573818710058, -296.2949690949762953, -198.8732915153567831 ) ) ;
#84379=CARTESIAN_POINT ( 'NONE',  ( -79.31113783129632111, -279.4853316204519160, -331.6563028085305405 ) ) ;
#84380=CARTESIAN_POINT ( 'NONE',  ( -40.80931946509393526, -272.1477909254060705, -196.1564042169583502 ) ) ;
#84381=CARTESIAN_POINT ( 'NONE',  ( -93.37565050710217918, -297.0869188970864911, -317.7865627103959127 ) ) ;
#84382=CARTESIAN_POINT ( 'NONE',  ( -37.83835201206461818, -299.1254603554876894, -197.0536871750575756 ) ) ;
#84384=CARTESIAN_POINT ( 'NONE',  ( -94.96305480293479206, -297.4715766353095319, -320.2231265894918124 ) ) ;
#84385=CARTESIAN_POINT ( 'NONE',  ( -30.66177028539085114, -296.1354297406613227, -195.1967136867763770 ) ) ;
#84386=CARTESIAN_POINT ( 'NONE',  ( 2.288803294583334758, -293.2495721843046681, -208.8738361416342002 ) ) ;
#84387=CARTESIAN_POINT ( 'NONE',  ( -95.56958125686577432, -289.7553819729196789, -225.3623537982682024 ) ) ;
#84389=CARTESIAN_POINT ( 'NONE',  ( 34.66195457170497463, -275.7012276121154173, -243.2502232539497413 ) ) ;
#84390=CARTESIAN_POINT ( 'NONE',  ( -105.8271387144993838, -297.2248862334024011, -244.8808399273111434 ) ) ;
#84391=CARTESIAN_POINT ( 'NONE',  ( -4.399904543953398139, -282.4639787289951300, -202.5734303699094596 ) ) ;
#84392=CARTESIAN_POINT ( 'NONE',  ( 10.52758371878726606, -279.3820119313264740, -210.6121339448463345 ) ) ;
#84394=CARTESIAN_POINT ( 'NONE',  ( -102.0157615342755548, -277.3531132128244963, -312.0585213817184922 ) ) ;
#84395=CARTESIAN_POINT ( 'NONE',  ( 24.26089512400363546, -281.2952303774416691, -309.9222180815027627 ) ) ;
#84396=CARTESIAN_POINT ( 'NONE',  ( 35.22200958904141288, -279.2998677720605087, -250.7026428831857743 ) ) ;
#84397=CARTESIAN_POINT ( 'NONE',  ( -19.10821555870619548, -272.8660219129529878, -199.0136997246420094 ) ) ;
#84398=CARTESIAN_POINT ( 'NONE',  ( -101.8537144878484071, -281.0651545844107773, -232.0094727065487348 ) ) ;
#84401=CARTESIAN_POINT ( 'NONE',  ( -75.25460777804273960, -295.7943235094953138, -204.4479841024782729 ) ) ;
#84402=CARTESIAN_POINT ( 'NONE',  ( -73.43371414927439389, -291.5868802612986315, -202.3288195381723256 ) ) ;
#84403=CARTESIAN_POINT ( 'NONE',  ( 37.87315669704598520, -277.5621275463726079, -271.1269236137998746 ) ) ;
#84404=CARTESIAN_POINT ( 'NONE',  ( -54.64900273838330236, -271.8295515904222270, -197.3853828235882872 ) ) ;
#84406=CARTESIAN_POINT ( 'NONE',  ( -95.15248760389202687, -285.8044239998201874, -319.0352866211200080 ) ) ;
#84409=CARTESIAN_POINT ( 'NONE',  ( 32.79333726643868374, -285.8988922467241878, -297.0768020882682094 ) ) ;
#84411=CARTESIAN_POINT ( 'NONE',  ( 17.36634659898984623, -293.0434494363104250, -319.3102177360651126 ) ) ;
#84412=CARTESIAN_POINT ( 'NONE',  ( 30.54519158094267794, -286.0907552523072468, -300.5257973592997018 ) ) ;
#84413=CARTESIAN_POINT ( 'NONE',  ( -111.2639016180397959, -258.5489101121608542, -316.4159311957783984 ) ) ;
#84414=CARTESIAN_POINT ( 'NONE',  ( -61.68578411627769498, -293.3681722875534774, -341.3553400149617119 ) ) ;
#84415=CARTESIAN_POINT ( 'NONE',  ( -64.28411274121526731, -284.1867824856522589, -198.9551040473461399 ) ) ;
#84416=CARTESIAN_POINT ( 'NONE',  ( -83.95867758776994094, -280.9998560703292583, -213.0822174579490138 ) ) ;
#84417=CARTESIAN_POINT ( 'NONE',  ( 22.67118288217023192, -288.1166077668377739, -222.7328368943534826 ) ) ;
#84418=CARTESIAN_POINT ( 'NONE',  ( 5.629903472503285933, -278.8654579711358110, -207.6920243571024969 ) ) ;
#84419=CARTESIAN_POINT ( 'NONE',  ( -100.3039510493918698, -290.0436982626653162, -307.4032692991129920 ) ) ;
#84420=CARTESIAN_POINT ( 'NONE',  ( -83.82386135046982645, -280.8250281173230292, -213.2444390358841417 ) ) ;
#84421=CARTESIAN_POINT ( 'NONE',  ( 26.59500856852853801, -281.8698230888882676, -234.7985111099180244 ) ) ;
#84422=CARTESIAN_POINT ( 'NONE',  ( -32.43915910271285696, -288.0935410092928919, -195.1526751699746853 ) ) ;
#84424=CARTESIAN_POINT ( 'NONE',  ( -64.90008180760548839, -273.7019828982753324, -198.4474496965166850 ) ) ;
#84425=CARTESIAN_POINT ( 'NONE',  ( -109.9444822227654726, -292.3083154189519064, -287.7013267156555116 ) ) ;
#84427=CARTESIAN_POINT ( 'NONE',  ( 25.22466315766300227, -296.6948066931273047, -320.2154176792147382 ) ) ;
#84429=CARTESIAN_POINT ( 'NONE',  ( -46.62862727319261325, -271.9343522624728848, -195.7703584392898506 ) ) ;
#84431=CARTESIAN_POINT ( 'NONE',  ( -6.144064501548008650, -293.0488659797035211, -339.8819634091275930 ) ) ;
#84432=CARTESIAN_POINT ( 'NONE',  ( -109.9861389561575606, -272.0083040098116385, -262.1954474380292481 ) ) ;
#84433=CARTESIAN_POINT ( 'NONE',  ( -85.11996740817369300, -291.2455956538783539, -326.5350072438603775 ) ) ;
#84434=CARTESIAN_POINT ( 'NONE',  ( -64.40532340248850574, -285.1704349223907684, -339.2489565985646891 ) ) ;
#84435=CARTESIAN_POINT ( 'NONE',  ( -67.80218318753259155, -290.8694452443189107, -340.4379705508233656 ) ) ;
#84436=CARTESIAN_POINT ( 'NONE',  ( -80.25009160482950676, -290.9348400447664176, -333.7667869390358533 ) ) ;
#84437=CARTESIAN_POINT ( 'NONE',  ( 1.174480116851917000, -288.5661438619765704, -205.9460609092934362 ) ) ;
#84438=CARTESIAN_POINT ( 'NONE',  ( 20.12727118129029336, -281.0238504726803512, -219.0936848592017725 ) ) ;
#84439=CARTESIAN_POINT ( 'NONE',  ( -92.65236900269162845, -293.9167738930667042, -321.8587601983239210 ) ) ;
#84440=CARTESIAN_POINT ( 'NONE',  ( -96.27168324184222570, -283.7179273768416579, -319.9421601307173546 ) ) ;
#84441=CARTESIAN_POINT ( 'NONE',  ( 10.25926550139060112, -276.5769256824539184, -213.3287994548637698 ) ) ;
#84442=CARTESIAN_POINT ( 'NONE',  ( -82.13390479932378696, -281.9090924074130839, -214.2458315076590907 ) ) ;
#84443=CARTESIAN_POINT ( 'NONE',  ( 7.623145230536814587, -274.6881534806597642, -331.6809371522889478 ) ) ;
#84445=CARTESIAN_POINT ( 'NONE',  ( 34.54487186711776303, -281.2327362140775904, -283.4814450499389409 ) ) ;
#84446=CARTESIAN_POINT ( 'NONE',  ( -56.80823074348885626, -278.5026900084931754, -344.5040937399404015 ) ) ;
#84447=CARTESIAN_POINT ( 'NONE',  ( -73.49157915535057839, -284.6436272365019136, -202.5821886492836654 ) ) ;
#84448=CARTESIAN_POINT ( 'NONE',  ( 32.75359282100029645, -294.9990178746637639, -246.4399053763661414 ) ) ;
#84449=CARTESIAN_POINT ( 'NONE',  ( -16.02093885647730787, -275.9233740138575968, -197.1499131875742989 ) ) ;
#84450=CARTESIAN_POINT ( 'NONE',  ( -44.01653318996780939, -275.2847446179963526, -194.0930282987283135 ) ) ;
#84452=CARTESIAN_POINT ( 'NONE',  ( -3.869357443563839816, -276.4309700254543714, -335.2348590473265517 ) ) ;
#84453=CARTESIAN_POINT ( 'NONE',  ( -66.75074450077376298, -297.4385148179549674, -339.1734463673220148 ) ) ;
#84454=CARTESIAN_POINT ( 'NONE',  ( -42.78263105986803083, -283.9831991596627745, -195.7128974807595512 ) ) ;
#84455=CARTESIAN_POINT ( 'NONE',  ( -13.86886206668244625, -292.0151998331343179, -196.9923333276430242 ) ) ;
#84456=CARTESIAN_POINT ( 'NONE',  ( 22.82150868883725536, -272.9668845987543477, -226.1770132627099485 ) ) ;
#84457=CARTESIAN_POINT ( 'NONE',  ( 25.20682555546215653, -289.7344516070701275, -313.9732632313541103 ) ) ;
#84458=CARTESIAN_POINT ( 'NONE',  ( 32.92932022341919662, -292.1951591364924070, -249.3004424128461380 ) ) ;
#84460=CARTESIAN_POINT ( 'NONE',  ( 17.08276957223457870, -291.3839738596577718, -216.6528036534279806 ) ) ;
#84461=CARTESIAN_POINT ( 'NONE',  ( -96.57825259539474416, -289.6219187260157355, -313.0591078487359482 ) ) ;
#84463=CARTESIAN_POINT ( 'NONE',  ( 23.05257439262340569, -289.2663167028348425, -317.6477320227812129 ) ) ;
#84464=CARTESIAN_POINT ( 'NONE',  ( -101.8736270309984633, -278.4200904000175001, -304.5330055055263756 ) ) ;
#84465=CARTESIAN_POINT ( 'NONE',  ( -11.17565106643310813, -293.6394588670135022, -342.5065009999817676 ) ) ;
#84466=CARTESIAN_POINT ( 'NONE',  ( -112.2622961920221627, -285.4205458410303322, -253.0343446932441509 ) ) ;
#84468=CARTESIAN_POINT ( 'NONE',  ( -52.17336884950474030, -286.2006795055660859, -194.7702219466202678 ) ) ;
#84469=CARTESIAN_POINT ( 'NONE',  ( -13.51845849879097727, -283.0675675113317311, -339.4403912660196170 ) ) ;
#84470=CARTESIAN_POINT ( 'NONE',  ( 197.6044253294050463, 285.2818546706590723, -111.8431199949838799 ) ) ;
#84471=CARTESIAN_POINT ( 'NONE',  ( -114.3334731447618964, -272.3709480647709711, -270.3588108202161493 ) ) ;
#84472=CARTESIAN_POINT ( 'NONE',  ( -111.8583052612683559, -270.4238486108535540, -283.6505382273211922 ) ) ;
#84473=CARTESIAN_POINT ( 'NONE',  ( 25.41959993401218654, -274.2321322206071272, -232.6648183996918249 ) ) ;
#84474=CARTESIAN_POINT ( 'NONE',  ( 33.19152039684580302, -274.7360800206804470, -290.3892892549357612 ) ) ;
#84475=CARTESIAN_POINT ( 'NONE',  ( -113.1443483155298111, -295.8911790799460846, -283.8337008503282277 ) ) ;
#84476=CARTESIAN_POINT ( 'NONE',  ( -20.49356206675482994, -109.5565994813256907, -359.6110413397351522 ) ) ;
#84477=CARTESIAN_POINT ( 'NONE',  ( 18.53154563780501718, -274.9544382816224015, -322.6246681904901266 ) ) ;
#84478=CARTESIAN_POINT ( 'NONE',  ( 53.54104891564487900, -301.0620212793358519, -196.0967531908359263 ) ) ;
#84480=CARTESIAN_POINT ( 'NONE',  ( -91.47810984396089395, -298.2452671211477195, -215.9362215132393601 ) ) ;
#84482=CARTESIAN_POINT ( 'NONE',  ( 33.76242309124552321, -288.2659274682625323, -287.1596924186707156 ) ) ;
#84483=CARTESIAN_POINT ( 'NONE',  ( -34.84961870311571630, -295.8244189115176823, -347.1592192034344748 ) ) ;
#84484=CARTESIAN_POINT ( 'NONE',  ( -103.7998126312026841, -297.5505082227326170, -231.4895506836044774 ) ) ;
#84485=CARTESIAN_POINT ( 'NONE',  ( 32.34743403496987924, -294.0068588261889886, -292.0964483023908542 ) ) ;
#84488=CARTESIAN_POINT ( 'NONE',  ( 37.49453677952599406, -277.3393367683453334, -259.9279093017450464 ) ) ;
#84491=ORIENTED_EDGE ( 'NONE', *, *, #75831, .F. ) ;
#84492=CARTESIAN_POINT ( 'NONE',  ( 26.23330936383726808, -280.4867806933232828, -226.9351918812147346 ) ) ;
#84493=CARTESIAN_POINT ( 'NONE',  ( -3.748893341467848028, -277.5387228653668785, -335.4374714524922183 ) ) ;
#84494=CARTESIAN_POINT ( 'NONE',  ( 13.27257980712055918, -276.5082649256934815, -213.6148257675565958 ) ) ;
#84495=CARTESIAN_POINT ( 'NONE',  ( -86.05162485144307993, -275.7431319580067566, -327.9250637786943230 ) ) ;
#84496=CARTESIAN_POINT ( 'NONE',  ( -63.12317116106024173, -298.3588455627964322, -201.9028211954180563 ) ) ;
#84497=CARTESIAN_POINT ( 'NONE',  ( -109.4658248454135787, -294.9348528856303915, -285.0350917772594244 ) ) ;
#84499=CARTESIAN_POINT ( 'NONE',  ( -8.889701417104502568, -280.9068756044500788, -198.8767793298676168 ) ) ;
#84500=CARTESIAN_POINT ( 'NONE',  ( -11.25205911331266506, -276.8691436503701198, -338.5397849996453488 ) ) ;
#84501=CARTESIAN_POINT ( 'NONE',  ( 23.47965045459499223, -285.6139985952347615, -223.9277635034149512 ) ) ;
#84502=CARTESIAN_POINT ( 'NONE',  ( -92.33917107632198906, -299.2684638623280193, -219.0474211882446127 ) ) ;
#84504=CARTESIAN_POINT ( 'NONE',  ( -5.731900617721290558, -287.8226513021683104, -336.3415870812905268 ) ) ;
#84505=CARTESIAN_POINT ( 'NONE',  ( 3.278600209230730034, -278.8456605912011810, -208.4290573766685952 ) ) ;
#84506=CARTESIAN_POINT ( 'NONE',  ( -19.37325337634339206, -278.8624451049915933, -198.9465788586520603 ) ) ;
#84507=CARTESIAN_POINT ( 'NONE',  ( -100.2610150942315670, -282.0918041885346952, -310.2379879165210923 ) ) ;
#84508=CARTESIAN_POINT ( 'NONE',  ( 5.473358113971913852, -288.6315135154992504, -208.7207170677915826 ) ) ;
#84509=CARTESIAN_POINT ( 'NONE',  ( -93.40337145249286266, -280.4269895856880908, -222.9685858626709773 ) ) ;
#84511=CARTESIAN_POINT ( 'NONE',  ( -28.12091379636063238, -294.1692172861027643, -195.8778125691332264 ) ) ;
#84512=CARTESIAN_POINT ( 'NONE',  ( -67.32960535011552849, -275.6799215561296705, -340.1801666420981292 ) ) ;
#84513=CARTESIAN_POINT ( 'NONE',  ( -18.98334697238140123, -277.4609261147664938, -341.1203119947492723 ) ) ;
#84514=CARTESIAN_POINT ( 'NONE',  ( 17.79756720892234512, -282.8394078394411508, -219.2759966199120640 ) ) ;
#84515=CARTESIAN_POINT ( 'NONE',  ( 145.2857639756989272, -299.5541904835127980, -195.3611179825600175 ) ) ;
#84516=CARTESIAN_POINT ( 'NONE',  ( -43.04867894218896396, -291.0438270114022998, -345.7052922174098057 ) ) ;
#84517=CARTESIAN_POINT ( 'NONE',  ( -23.10655727017623917, -292.8700466203845849, -344.0501218334949840 ) ) ;
#84518=CARTESIAN_POINT ( 'NONE',  ( -83.17135601502684494, -284.6398509438687938, -208.6198081705028642 ) ) ;
#84520=CARTESIAN_POINT ( 'NONE',  ( -79.12175298627666109, -272.1605615289080333, -209.8371671954822375 ) ) ;
#84521=CARTESIAN_POINT ( 'NONE',  ( -34.79151669280420123, -290.2241130347376838, -196.1697300255089829 ) ) ;
#84524=CARTESIAN_POINT ( 'NONE',  ( -41.99219267714649817, -290.4744182489737909, -194.1962922932764570 ) ) ;
#84525=CARTESIAN_POINT ( 'NONE',  ( -23.94227290191253132, -284.4607735636431016, -195.5116938786316894 ) ) ;
#84526=CARTESIAN_POINT ( 'NONE',  ( -110.8177567921373878, -286.0417802461519727, -265.4437703624051892 ) ) ;
#84527=CARTESIAN_POINT ( 'NONE',  ( 2.526466785016224126, -287.4046897439871486, -209.0167539895106756 ) ) ;
#84528=CARTESIAN_POINT ( 'NONE',  ( 14.29238269885748380, -294.7529144959206633, -215.4048136358007923 ) ) ;
#84530=CARTESIAN_POINT ( 'NONE',  ( 29.26198385745171038, -274.1032667765052793, -306.1543468366396610 ) ) ;
#84531=CARTESIAN_POINT ( 'NONE',  ( 38.19718175543830796, -275.7000407672019833, -255.5414818402107358 ) ) ;
#84532=CARTESIAN_POINT ( 'NONE',  ( -2.693939750755892426, -290.5864108989727015, -203.1986668263294007 ) ) ;
#84533=CARTESIAN_POINT ( 'NONE',  ( -95.90580814570735413, -279.2266411864729321, -220.3484144840087424 ) ) ;
#84534=CARTESIAN_POINT ( 'NONE',  ( -109.5545231652896661, -298.2874343649134516, -289.3101322593834652 ) ) ;
#84537=CARTESIAN_POINT ( 'NONE',  ( -96.96516594762569241, -283.8340900648736920, -227.3712274558124307 ) ) ;
#84538=CARTESIAN_POINT ( 'NONE',  ( -97.80014055207578849, -277.1574277957417962, -225.9572756666332225 ) ) ;
#84540=CARTESIAN_POINT ( 'NONE',  ( -18.70044056565021862, -272.7677251476854963, -196.3119100973368631 ) ) ;
#84541=CARTESIAN_POINT ( 'NONE',  ( -40.51848743638214501, -276.4417018124065066, -343.4064736804778022 ) ) ;
#84542=CARTESIAN_POINT ( 'NONE',  ( -10.21696186102800930, -296.2116682201667572, -338.8808693452598959 ) ) ;
#84543=CARTESIAN_POINT ( 'NONE',  ( -3.780416096598072873, -279.4049107028315007, -201.3891861335980309 ) ) ;
#84544=CARTESIAN_POINT ( 'NONE',  ( -12.91851203659506453, -295.6682028422287090, -339.4574100867980633 ) ) ;
#84545=CARTESIAN_POINT ( 'NONE',  ( -105.5106409123517039, -297.4158461493966570, -305.2095094465364014 ) ) ;
#84546=CARTESIAN_POINT ( 'NONE',  ( -98.44640764112762099, -296.9400876153848685, -230.3295074395100528 ) ) ;
#84547=CARTESIAN_POINT ( 'NONE',  ( -80.70733034375930970, -293.4645102605961142, -209.1057582158795753 ) ) ;
#84548=CARTESIAN_POINT ( 'NONE',  ( -67.19101861561325961, -285.8381280934745519, -199.3821197482443495 ) ) ;
#84549=CARTESIAN_POINT ( 'NONE',  ( 37.51103972702107825, -273.5417016604889113, -258.5567114111759679 ) ) ;
#84550=CARTESIAN_POINT ( 'NONE',  ( -68.05582737115803127, -289.2777502104871132, -340.9701994963284051 ) ) ;
#84551=CARTESIAN_POINT ( 'NONE',  ( -21.87773377124138108, -282.2310454560187054, -197.2826716088150647 ) ) ;
#84553=CARTESIAN_POINT ( 'NONE',  ( -17.09536289837461709, -285.3786407768920981, -199.9270325773222510 ) ) ;
#84554=CARTESIAN_POINT ( 'NONE',  ( -72.47371337224363685, -289.5870430560574960, -204.0839309381270255 ) ) ;
#84555=CARTESIAN_POINT ( 'NONE',  ( -87.71122462277782006, -229.8683413793775117, -344.1918058839762011 ) ) ;
#84556=CARTESIAN_POINT ( 'NONE',  ( -8.224665675238146179, -285.9517117804990107, -203.3522622508393738 ) ) ;
#84558=CARTESIAN_POINT ( 'NONE',  ( 34.37197863709827317, -282.8411621796157647, -297.7466705684454951 ) ) ;
#84559=CARTESIAN_POINT ( 'NONE',  ( -111.7634962471925917, -289.8477185536031016, -251.4875653462070773 ) ) ;
#84560=CARTESIAN_POINT ( 'NONE',  ( -40.99068555384094736, -281.6071083202118075, -194.2354764654441226 ) ) ;
#84561=CARTESIAN_POINT ( 'NONE',  ( -108.1933901517096359, -279.4983224362807732, -299.2286826949339797 ) ) ;
#84562=CARTESIAN_POINT ( 'NONE',  ( 32.73518496775560749, -281.1149334008352412, -249.9104412265337487 ) ) ;
#84563=CARTESIAN_POINT ( 'NONE',  ( 36.12877936576951043, -277.7458007121079504, -285.4306002317723596 ) ) ;
#84564=CARTESIAN_POINT ( 'NONE',  ( 22.28663472010287805, -294.2063025763596329, -319.1000031672770092 ) ) ;
#84565=CARTESIAN_POINT ( 'NONE',  ( -78.13338405222577876, -289.5207895896929813, -207.8480367620082916 ) ) ;
#84566=CARTESIAN_POINT ( 'NONE',  ( -109.5173458489569498, -271.5255873135467937, -256.7551377422548740 ) ) ;
#84569=CARTESIAN_POINT ( 'NONE',  ( -111.0412837155565740, -286.6077944729850628, -259.8880297537694446 ) ) ;
#84570=CARTESIAN_POINT ( 'NONE',  ( -102.7889931746739904, -295.7786440147611984, -302.8596403196340816 ) ) ;
#84571=CARTESIAN_POINT ( 'NONE',  ( 24.55680202845721993, -294.0282434784202792, -225.0834420132484013 ) ) ;
#84572=CARTESIAN_POINT ( 'NONE',  ( -18.70164910337568642, -283.4572461733512796, -341.0991058558648206 ) ) ;
#84573=CARTESIAN_POINT ( 'NONE',  ( -24.18809762182304723, -273.2747913133352995, -194.6777368749933146 ) ) ;
#84574=CARTESIAN_POINT ( 'NONE',  ( -113.0730773364861932, -291.3706731435830193, -257.0167823721474747 ) ) ;
#84575=CARTESIAN_POINT ( 'NONE',  ( -46.33499748532583595, -284.0787806046485002, -195.1319608569893660 ) ) ;
#84576=CARTESIAN_POINT ( 'NONE',  ( -44.89919570228643408, -292.2923718770568939, -193.7012355447725724 ) ) ;
#84577=CARTESIAN_POINT ( 'NONE',  ( 35.70139722419138195, -287.8583545154607464, -268.3076320364752405 ) ) ;
#84580=CARTESIAN_POINT ( 'NONE',  ( 179.5473848012214262, 251.1466290182995351, -164.2343626752925729 ) ) ;
#84581=CARTESIAN_POINT ( 'NONE',  ( 13.23584927058908534, -283.8805131436979536, -327.5683142627717075 ) ) ;
#84582=CARTESIAN_POINT ( 'NONE',  ( -20.19161114001082069, -283.7666405000204009, -195.3683826091709363 ) ) ;
#84584=CARTESIAN_POINT ( 'NONE',  ( 34.64037142633370081, -280.2892074466396366, -256.4094100199512241 ) ) ;
#84585=CARTESIAN_POINT ( 'NONE',  ( -11.87718457728808374, -276.3963940815153251, -343.0620742489219879 ) ) ;
#84586=CARTESIAN_POINT ( 'NONE',  ( -73.02580578515330956, -281.5781949007277944, -204.5836671965063545 ) ) ;
#84587=CARTESIAN_POINT ( 'NONE',  ( 104.8979029556089984, 114.3573006684971176, -281.0218342242372387 ) ) ;
#84588=CARTESIAN_POINT ( 'NONE',  ( 19.70100152600230103, -279.4321552419335717, -219.5011347623741642 ) ) ;
#84589=CARTESIAN_POINT ( 'NONE',  ( -71.91821957149345224, -283.6127663966410637, -204.2074248991358445 ) ) ;
#84590=CARTESIAN_POINT ( 'NONE',  ( -112.2015885280200393, -298.1433036508663577, -283.6952532771364872 ) ) ;
#84591=CARTESIAN_POINT ( 'NONE',  ( 19.38961205466062054, -293.3934677931824808, -224.3027988332710834 ) ) ;
#84593=CARTESIAN_POINT ( 'NONE',  ( -90.15917315633986107, -289.9705278726449365, -219.2577128042854895 ) ) ;
#84594=CARTESIAN_POINT ( 'NONE',  ( -51.28598297934721728, -277.8773621177044220, -345.9843271319578548 ) ) ;
#84595=CARTESIAN_POINT ( 'NONE',  ( -37.15174342076831238, -298.2212839986111703, -197.3582636486453339 ) ) ;
#84597=CARTESIAN_POINT ( 'NONE',  ( -44.00215429290172153, -272.8902854639284214, -193.9069058675410702 ) ) ;
#84599=CARTESIAN_POINT ( 'NONE',  ( 104.1964229570258311, -299.5541904835127980, -195.3611179825600175 ) ) ;
#84602=CARTESIAN_POINT ( 'NONE',  ( -29.39754862652458201, -284.0289769777061792, -343.2892433025422179 ) ) ;
#84603=CARTESIAN_POINT ( 'NONE',  ( -5.854689970467189752, -284.4039895035847962, -339.5170447559394802 ) ) ;
#84605=CARTESIAN_POINT ( 'NONE',  ( -110.5441588553734249, -283.6397285687048679, -268.1682924790215452 ) ) ;
#84606=CARTESIAN_POINT ( 'NONE',  ( -7.524701240498339772, -282.3076679480644202, -202.3633062496137143 ) ) ;
#84607=CARTESIAN_POINT ( 'NONE',  ( 7.991815190154221149, -274.8999062043310460, -328.5258709774581689 ) ) ;
#84609=CARTESIAN_POINT ( 'NONE',  ( 35.66308507941423755, -276.7194845221019364, -277.0340041590820874 ) ) ;
#84611=CARTESIAN_POINT ( 'NONE',  ( -96.92268435407343929, -278.7022862665535285, -318.9024891875315006 ) ) ;
#84615=CARTESIAN_POINT ( 'NONE',  ( -46.38199491702875576, -287.7990128282820592, -195.1375940734226901 ) ) ;
#84616=CARTESIAN_POINT ( 'NONE',  ( 10.38915617819067982, -293.5703017978193543, -325.8080933981307794 ) ) ;
#84618=CARTESIAN_POINT ( 'NONE',  ( -48.86192889167434572, -288.5436588147713906, -346.4452298758017150 ) ) ;
#84619=CARTESIAN_POINT ( 'NONE',  ( -88.37725866931455698, -283.5648368278256726, -216.7575194431497891 ) ) ;
#84620=CARTESIAN_POINT ( 'NONE',  ( -107.5534399211838377, -282.8371188648794146, -292.3994144810747571 ) ) ;
#84621=CARTESIAN_POINT ( 'NONE',  ( 4.164595750138585295, -286.7245440666101217, -331.7026040310582289 ) ) ;
#84622=CARTESIAN_POINT ( 'NONE',  ( -92.84941488616658489, -285.0764923312933661, -318.4013188499606031 ) ) ;
#84623=CARTESIAN_POINT ( 'NONE',  ( -6.140646871974609233, -274.6419973838914643, -338.5629869318368037 ) ) ;
#84624=CARTESIAN_POINT ( 'NONE',  ( 21.48569449982180046, -285.2945054122856732, -221.9278849769301871 ) ) ;
#84625=CARTESIAN_POINT ( 'NONE',  ( -111.4183016896326706, -298.7040071291575600, -258.5468238337924163 ) ) ;
#84626=CARTESIAN_POINT ( 'NONE',  ( -24.08362996353298868, -284.2207929286254284, -196.3200007184363187 ) ) ;
#84627=CARTESIAN_POINT ( 'NONE',  ( 13.48981789208581894, -281.7260268329336554, -217.5688768104170379 ) ) ;
#84628=CARTESIAN_POINT ( 'NONE',  ( -6.358348707647138554, -290.6462704121202592, -338.8451333783993391 ) ) ;
#84631=CARTESIAN_POINT ( 'NONE',  ( -6.365254188959164949, -296.5685791259637654, -339.2797221327722923 ) ) ;
#84632=CARTESIAN_POINT ( 'NONE',  ( -84.68092123261685344, -277.4001464960598469, -212.1217702207200944 ) ) ;
#84633=CARTESIAN_POINT ( 'NONE',  ( 21.19408760908437372, -292.0766276590422876, -220.5643083970942087 ) ) ;
#84634=CARTESIAN_POINT ( 'NONE',  ( -61.29184687826233358, -293.7681399212100359, -340.2209503814428899 ) ) ;
#84635=CARTESIAN_POINT ( 'NONE',  ( -81.57140323778570234, -278.1210370361632727, -211.6033012207521438 ) ) ;
#84636=CARTESIAN_POINT ( 'NONE',  ( -108.5673262555312562, -270.9150424210555457, -248.5462471325402305 ) ) ;
#84637=CARTESIAN_POINT ( 'NONE',  ( 22.98321295827224020, -294.2858875596326129, -228.3610005819590469 ) ) ;
#84638=CARTESIAN_POINT ( 'NONE',  ( -110.4542110544635705, -298.8376638359844719, -287.0812184334320705 ) ) ;
#84639=CARTESIAN_POINT ( 'NONE',  ( -105.8819918231437356, -295.4666606691158108, -236.8210499260000859 ) ) ;
#84640=CARTESIAN_POINT ( 'NONE',  ( 36.77791863643169989, -291.5791904114416297, -253.5618488223141469 ) ) ;
#84641=CARTESIAN_POINT ( 'NONE',  ( -91.01014542618868575, -291.2579636640669491, -320.7850197730614923 ) ) ;
#84643=CARTESIAN_POINT ( 'NONE',  ( -47.02593662354598791, -292.7288303693555349, -197.8434146943737062 ) ) ;
#84645=CARTESIAN_POINT ( 'NONE',  ( -104.2705418291623687, -292.2427898216975564, -233.0980147010666030 ) ) ;
#84646=CARTESIAN_POINT ( 'NONE',  ( 29.27970278240654523, -279.1063614056792517, -235.0362351616882108 ) ) ;
#84647=CARTESIAN_POINT ( 'NONE',  ( 20.18289337632174352, -292.9184244090254765, -225.3973482517065179 ) ) ;
#84648=CARTESIAN_POINT ( 'NONE',  ( -19.75622297167328512, -280.2720795538326115, -195.3413490507532799 ) ) ;
#84649=CARTESIAN_POINT ( 'NONE',  ( -96.25687101198548135, -283.5513531797032556, -319.9269173938301947 ) ) ;
#84650=CARTESIAN_POINT ( 'NONE',  ( -74.47631261130082692, -287.5470648378947089, -335.3454942629221023 ) ) ;
#84651=CARTESIAN_POINT ( 'NONE',  ( -32.08142562831677935, -281.1246676961565072, -344.4097168422595132 ) ) ;
#84652=CARTESIAN_POINT ( 'NONE',  ( -7.787486001178397288, -278.9123432563246752, -199.9959917526237803 ) ) ;
#84653=CARTESIAN_POINT ( 'NONE',  ( -54.88051069804145499, -284.7520938587618389, -195.7026781873072707 ) ) ;
#84655=CARTESIAN_POINT ( 'NONE',  ( -4.495127717372585430, -294.0924533125566995, -204.2596524295456391 ) ) ;
#84656=CARTESIAN_POINT ( 'NONE',  ( 32.01057792079404152, -276.5624367077597299, -238.1592124264664676 ) ) ;
#84657=CARTESIAN_POINT ( 'NONE',  ( -99.19526130156747001, -277.6819655194600500, -309.2656835814856322 ) ) ;
#84658=CARTESIAN_POINT ( 'NONE',  ( -110.7812034713324039, -290.4260214670683808, -293.6791763000610445 ) ) ;
#84659=CARTESIAN_POINT ( 'NONE',  ( 12.70830716631821389, -280.4407908647269778, -327.0373755569534069 ) ) ;
#84661=CARTESIAN_POINT ( 'NONE',  ( 34.71683709249455774, -292.4380423093900276, -257.2155570980069115 ) ) ;
#84662=CARTESIAN_POINT ( 'NONE',  ( -96.70741020440551949, -293.9239326537086754, -316.1946550473429056 ) ) ;
#84665=CARTESIAN_POINT ( 'NONE',  ( -12.23317364619639847, -291.8953423973540566, -201.6956025926079974 ) ) ;
#84667=AXIS2_PLACEMENT_3D ( 'NONE', #32678, #54434, #83306 ) ;
#84668=CARTESIAN_POINT ( 'NONE',  ( -82.13390479932374433, -281.1952119285918457, -326.4764044574609443 ) ) ;
#84669=CARTESIAN_POINT ( 'NONE',  ( -111.3918943636935808, -295.8673282966256011, -249.9314521311504791 ) ) ;
#84670=CARTESIAN_POINT ( 'NONE',  ( 38.18235643354120867, -279.6150285160001658, -264.3260240273204431 ) ) ;
#84673=CARTESIAN_POINT ( 'NONE',  ( -12.87735421558434545, -287.6787865930397743, -197.8711597050102853 ) ) ;
#84674=CARTESIAN_POINT ( 'NONE',  ( 35.12395899986310610, -287.5017736918570677, -279.1774807049368405 ) ) ;
#84675=CARTESIAN_POINT ( 'NONE',  ( -36.43843583764431315, -278.5607892142865012, -344.0615033695391958 ) ) ;
#84676=CARTESIAN_POINT ( 'NONE',  ( -56.24362834746958129, -293.3168239188995585, -342.6266243905814122 ) ) ;
#84677=CARTESIAN_POINT ( 'NONE',  ( -102.3467730436001801, -297.8358630124637898, -305.7491739687496874 ) ) ;
#84678=CARTESIAN_POINT ( 'NONE',  ( -108.6719543624020901, -277.5740315345138356, -253.0658776848339073 ) ) ;
#84681=CARTESIAN_POINT ( 'NONE',  ( -110.7808982374902911, -295.9283464484436763, -293.4796578382243410 ) ) ;
#84682=CARTESIAN_POINT ( 'NONE',  ( -109.7454457200876732, -292.2485869581113889, -287.6530763989714501 ) ) ;
#84684=CARTESIAN_POINT ( 'NONE',  ( 33.18245165197373581, -288.4596492910171719, -289.7905777935097831 ) ) ;
#84686=CARTESIAN_POINT ( 'NONE',  ( -40.98519899481389928, -279.0661385181588230, -193.6697707235305472 ) ) ;
#84687=CARTESIAN_POINT ( 'NONE',  ( -104.5098224891832643, -296.7162949563278289, -307.9099859867413898 ) ) ;
#84688=CARTESIAN_POINT ( 'NONE',  ( -112.8829774453177208, -288.6095878729155970, -276.8242574385814123 ) ) ;
#84690=CARTESIAN_POINT ( 'NONE',  ( -110.7942305705971080, -297.1769013780221371, -247.1524508713619355 ) ) ;
#84691=CARTESIAN_POINT ( 'NONE',  ( 33.66733163020020214, -293.6602690152835748, -253.2840564973251674 ) ) ;
#84695=CARTESIAN_POINT ( 'NONE',  ( 14.15025396002171831, -289.8650275804877197, -326.7469132408336918 ) ) ;
#84696=CARTESIAN_POINT ( 'NONE',  ( -88.47809603358389552, -280.1948066931273615, -334.5364918783848793 ) ) ;
#84697=EDGE_LOOP ( 'NONE', ( #17315, #41812, #9066, #42317 ) ) ;
#84698=CARTESIAN_POINT ( 'NONE',  ( 20.99419836792590388, -280.2234051625807183, -220.2388400288934918 ) ) ;
#84699=CARTESIAN_POINT ( 'NONE',  ( -63.22018972664060499, -287.7145853112636473, -200.0895239626313469 ) ) ;
#84700=CARTESIAN_POINT ( 'NONE',  ( 24.23925055052949773, -285.5213923579242987, -225.1240446071109602 ) ) ;
#84701=CARTESIAN_POINT ( 'NONE',  ( -93.37441368050792789, -271.2433656057248754, -220.7590672161392717 ) ) ;
#84702=CARTESIAN_POINT ( 'NONE',  ( -46.37734614304641667, -275.8567679110998370, -196.4715294218481461 ) ) ;
#84703=CARTESIAN_POINT ( 'NONE',  ( -83.45712644497612587, -287.7699418104172651, -328.7963954310883423 ) ) ;
#84704=CARTESIAN_POINT ( 'NONE',  ( -112.4950573596744334, -280.5397487875893603, -260.3548702983563885 ) ) ;
#84706=CARTESIAN_POINT ( 'NONE',  ( -81.28787849535682142, -279.4359994262300120, -212.0075647879850465 ) ) ;
#84707=CARTESIAN_POINT ( 'NONE',  ( 34.16664434493925029, -280.7000024331819645, -255.1208841223880484 ) ) ;
#84708=CARTESIAN_POINT ( 'NONE',  ( 16.74700613502275104, -277.3841904788619672, -324.8035154789374133 ) ) ;
#84709=CARTESIAN_POINT ( 'NONE',  ( -111.3434381929979082, -277.5967651603709214, -250.5178024289012058 ) ) ;
#84710=CARTESIAN_POINT ( 'NONE',  ( -23.38302767679204308, -107.9165556172637537, -359.8680264726103246 ) ) ;
#84711=CARTESIAN_POINT ( 'NONE',  ( -112.2164470930137981, -273.7057689388974495, -253.4320754468055839 ) ) ;
#84712=CARTESIAN_POINT ( 'NONE',  ( -112.3900044434635817, -274.2499993953724129, -256.2779135276613829 ) ) ;
#84713=CARTESIAN_POINT ( 'NONE',  ( -95.95921662488163406, -286.4090924074130839, -317.1477375740089997 ) ) ;
#84715=CARTESIAN_POINT ( 'NONE',  ( 34.31574213812709218, -288.8358157354460900, -285.8937989022575152 ) ) ;
#84716=CARTESIAN_POINT ( 'NONE',  ( 27.81790765058295634, -288.7944951500990101, -231.1674942962002604 ) ) ;
#84717=CARTESIAN_POINT ( 'NONE',  ( -108.4515006946262616, -289.6774359606176290, -287.3107177402468437 ) ) ;
#84718=CARTESIAN_POINT ( 'NONE',  ( -83.85099562316381139, -283.1789729676905267, -331.7176246685296519 ) ) ;
#84719=CARTESIAN_POINT ( 'NONE',  ( -57.31031176507513436, -278.1899923617590957, -199.3139860024720633 ) ) ;
#84720=CARTESIAN_POINT ( 'NONE',  ( -86.56256127943112233, -287.2205351154871096, -214.7210659250795288 ) ) ;
#84721=CARTESIAN_POINT ( 'NONE',  ( 36.38145335926363089, -280.0088260779004372, -268.5860096695554375 ) ) ;
#84722=CARTESIAN_POINT ( 'NONE',  ( -74.77127618962455813, -280.8582199984024896, -207.0549270406785354 ) ) ;
#84723=CARTESIAN_POINT ( 'NONE',  ( -1.434521781129437512, -277.0549926395453326, -334.0474746989127084 ) ) ;
#84724=CARTESIAN_POINT ( 'NONE',  ( 28.55431942628628761, -286.8586337448199970, -309.4216264878447191 ) ) ;
#84725=CARTESIAN_POINT ( 'NONE',  ( -10.74830540271383228, -283.5169672535341761, -342.5075242484209070 ) ) ;
#84726=CARTESIAN_POINT ( 'NONE',  ( -95.28425453745306584, -284.3593478299513890, -320.9791710059241723 ) ) ;
#84727=CARTESIAN_POINT ( 'NONE',  ( -16.13047405776010024, -282.9367921103295203, -340.2115574449022120 ) ) ;
#84730=CARTESIAN_POINT ( 'NONE',  ( -106.1487629417414098, -292.8263129146864117, -238.5202094795858443 ) ) ;
#84731=CARTESIAN_POINT ( 'NONE',  ( -22.27441263933424409, -290.9259218194210348, -195.2986374772053466 ) ) ;
#84732=CARTESIAN_POINT ( 'NONE',  ( -11.39567996390432292, -273.4572536321517759, -201.8217678506137531 ) ) ;
#84733=CARTESIAN_POINT ( 'NONE',  ( 19.44879114161051703, -293.6072841746498057, -322.2860680568882685 ) ) ;
#84735=CARTESIAN_POINT ( 'NONE',  ( -105.7639325553857645, -288.6675410030409807, -297.8679640479024897 ) ) ;
#84736=CARTESIAN_POINT ( 'NONE',  ( 34.94427830642977995, -291.5844112301731457, -254.4055386044406646 ) ) ;
#84737=CARTESIAN_POINT ( 'NONE',  ( -109.3251579806793075, -291.5682997801242209, -284.7610372288885401 ) ) ;
#84739=CARTESIAN_POINT ( 'NONE',  ( -109.6078751263233784, -292.2942188588540375, -290.4260276988350711 ) ) ;
#84740=CARTESIAN_POINT ( 'NONE',  ( 30.54150309095506799, -291.1267789772827541, -237.9616072299320138 ) ) ;
#84742=CARTESIAN_POINT ( 'NONE',  ( 36.88765235938980425, -295.6911480231632368, -281.1738630368813574 ) ) ;
#84743=CARTESIAN_POINT ( 'NONE',  ( -33.23741947741860514, -287.0462135641232067, -197.1909391565655199 ) ) ;
#84744=CARTESIAN_POINT ( 'NONE',  ( 26.56108238362537932, -296.0836441875538299, -310.0375213366009461 ) ) ;
#84745=CARTESIAN_POINT ( 'NONE',  ( 34.16107026347832232, -277.2241827566902543, -246.4110790618088629 ) ) ;
#84746=CARTESIAN_POINT ( 'NONE',  ( -99.78435095805376420, -296.3439619059403185, -225.5830633345405545 ) ) ;
#84747=CARTESIAN_POINT ( 'NONE',  ( 36.10887726020285982, -273.9158375105640175, -279.8785685496325186 ) ) ;
#84748=CARTESIAN_POINT ( 'NONE',  ( -54.80738866751382687, -277.9058833096234480, -197.9458621699358787 ) ) ;
#84749=CARTESIAN_POINT ( 'NONE',  ( -92.32574634542643821, -274.4480840224735516, -221.7413157714183569 ) ) ;
#84750=CARTESIAN_POINT ( 'NONE',  ( -110.3230004952766166, -298.1060029764889237, -260.5359188559763766 ) ) ;
#84752=CARTESIAN_POINT ( 'NONE',  ( -77.60936398729224095, -298.2995312104695813, -209.2173654003723016 ) ) ;
#84754=CARTESIAN_POINT ( 'NONE',  ( 31.22608769093933745, -285.1625677516429960, -238.9805696521124503 ) ) ;
#84755=CARTESIAN_POINT ( 'NONE',  ( 94.40996231196450594, -299.7467194292196382, -197.3612517501071864 ) ) ;
#84756=CARTESIAN_POINT ( 'NONE',  ( -36.56543202773214318, -286.0616424611802131, -193.3519920686951536 ) ) ;
#84757=CARTESIAN_POINT ( 'NONE',  ( -103.7823230088408479, -289.7115626355816289, -309.3431339259833521 ) ) ;
#84758=CARTESIAN_POINT ( 'NONE',  ( -94.34380924369031618, -299.2129856554471417, -220.9966340517623564 ) ) ;
#84759=CARTESIAN_POINT ( 'NONE',  ( -2.307449892412390735, -292.5872080995020497, -336.4869808458252578 ) ) ;
#84760=CARTESIAN_POINT ( 'NONE',  ( 22.75543048566671800, -280.1067417238356256, -222.4602033218193924 ) ) ;
#84761=CARTESIAN_POINT ( 'NONE',  ( -54.49178911615187815, -292.7666405000204577, -345.3538533559490702 ) ) ;
#84762=CARTESIAN_POINT ( 'NONE',  ( -112.2682631038234575, -276.6075373647698825, -266.0347761404772200 ) ) ;
#84763=CARTESIAN_POINT ( 'NONE',  ( -0.8070456546349069615, -287.3506722593737095, -334.0776805057863044 ) ) ;
#84765=CARTESIAN_POINT ( 'NONE',  ( -10.01859092377965865, -286.6953941853980155, -340.2627007679978988 ) ) ;
#84766=CARTESIAN_POINT ( 'NONE',  ( -108.6156099153904933, -274.3195619663922002, -251.4372613403305650 ) ) ;
#84767=CARTESIAN_POINT ( 'NONE',  ( 4.240385071979641651, -283.9290616604112643, -334.5293289439453019 ) ) ;
#84768=CARTESIAN_POINT ( 'NONE',  ( -32.02832856230393332, -296.1384645152230064, -195.0076918465410643 ) ) ;
#84769=CARTESIAN_POINT ( 'NONE',  ( 31.35459803861290240, -281.8828075987588022, -295.2050829412053758 ) ) ;
#84770=CARTESIAN_POINT ( 'NONE',  ( -105.9567382910251041, -296.2675369939992720, -305.4210399779860268 ) ) ;
#84771=CARTESIAN_POINT ( 'NONE',  ( -93.37414077111203881, -274.6506805554784592, -222.6369382647161217 ) ) ;
#84772=CARTESIAN_POINT ( 'NONE',  ( 37.92269054352076552, -285.5397119971207758, -263.1200446917670774 ) ) ;
#84773=CARTESIAN_POINT ( 'NONE',  ( 33.43170347536704412, -283.2290831294160398, -245.3842730494966702 ) ) ;
#84774=CARTESIAN_POINT ( 'NONE',  ( -33.78576006705885248, -297.1564869643439124, -197.1264078654978107 ) ) ;
#84777=CARTESIAN_POINT ( 'NONE',  ( -111.8721599483374689, -286.5963108412518636, -265.3800139427193585 ) ) ;
#84779=CARTESIAN_POINT ( 'NONE',  ( 13.84574458161073807, -278.1952119285919025, -206.2264541496106460 ) ) ;
#84780=CARTESIAN_POINT ( 'NONE',  ( 37.43235747293748261, -274.9717021062375579, -288.1095405543710513 ) ) ;
#84783=CARTESIAN_POINT ( 'NONE',  ( -99.60657900625787420, -285.5315257133872819, -309.8747869485899287 ) ) ;
#84784=CARTESIAN_POINT ( 'NONE',  ( 1.307565994427088985, -278.1271181248552580, -333.2914747882579718 ) ) ;
#84785=CARTESIAN_POINT ( 'NONE',  ( -111.1567905624018096, -286.2288391469839439, -250.4152047535799284 ) ) ;
#84786=CARTESIAN_POINT ( 'NONE',  ( -24.00833709386140313, -281.6729526445915326, -342.5369583582279347 ) ) ;
#84787=CARTESIAN_POINT ( 'NONE',  ( -4.710738447983236377, -282.4821269235096111, -202.8317096219167013 ) ) ;
#84788=CARTESIAN_POINT ( 'NONE',  ( -64.90206425053058581, -273.8686360474692378, -198.4482093745783686 ) ) ;
#84789=CARTESIAN_POINT ( 'NONE',  ( 14.88162004000146688, -276.1737655366200102, -327.0174710811662635 ) ) ;
#84790=CARTESIAN_POINT ( 'NONE',  ( -25.96364965714505857, -296.8262925768906939, -343.9264234137226595 ) ) ;
#84793=CARTESIAN_POINT ( 'NONE',  ( -108.2893624237504469, -294.3482952930792749, -297.0937443386634413 ) ) ;
#84794=CARTESIAN_POINT ( 'NONE',  ( -9.971123134216737682, -276.1925234148372397, -338.1156714925178903 ) ) ;
#84796=CARTESIAN_POINT ( 'NONE',  ( -55.01980313128539990, -287.5820087059923935, -198.4369648561895758 ) ) ;
#84797=CARTESIAN_POINT ( 'NONE',  ( 37.92563509238276964, -295.2316685289459315, -282.9917432509762421 ) ) ;
#84798=CARTESIAN_POINT ( 'NONE',  ( 39.25836179704051432, -294.7204588572359398, -267.4363748337179345 ) ) ;
#84799=CARTESIAN_POINT ( 'NONE',  ( -109.5269139884052834, -292.8066095119255010, -250.6298400540872819 ) ) ;
#84800=CARTESIAN_POINT ( 'NONE',  ( -77.79194998776431191, -277.5077983818829921, -207.3405966366347855 ) ) ;
#84801=CARTESIAN_POINT ( 'NONE',  ( -93.30690106862569166, -281.1594645595143902, -221.2580104515446919 ) ) ;
#84802=CARTESIAN_POINT ( 'NONE',  ( -39.75983852277892083, -293.1625717972547704, -344.7745111140371250 ) ) ;
#84803=CARTESIAN_POINT ( 'NONE',  ( -80.83282669348670879, -285.4954627753491536, -332.4638488983590605 ) ) ;
#84804=CARTESIAN_POINT ( 'NONE',  ( -98.35675271117310103, -284.0342402880223176, -229.7238268332223470 ) ) ;
#84805=CARTESIAN_POINT ( 'NONE',  ( 195.6780093180179563, 277.3413982316666875, -125.4371938877353898 ) ) ;
#84807=CARTESIAN_POINT ( 'NONE',  ( -108.7416330140586638, -284.0162923708891185, -285.7220592454714847 ) ) ;
#84809=CARTESIAN_POINT ( 'NONE',  ( 15.55032856930039742, -283.4044780371802972, -325.8942235091454904 ) ) ;
#84810=CARTESIAN_POINT ( 'NONE',  ( -91.61080955759018707, -284.0945860664872953, -216.2975213594836816 ) ) ;
#84811=CARTESIAN_POINT ( 'NONE',  ( -77.38005555113339540, -280.4706140308082354, -204.8033902624935365 ) ) ;
#84812=CARTESIAN_POINT ( 'NONE',  ( -37.10946225639649754, -278.5693742099411452, -346.6803751457239855 ) ) ;
#84813=CARTESIAN_POINT ( 'NONE',  ( -68.63864484960069490, -280.3029480464213066, -200.1056368983956304 ) ) ;
#84814=CARTESIAN_POINT ( 'NONE',  ( -37.30987171927208834, -271.5523547857346784, -200.3611179825600459 ) ) ;
#84815=CARTESIAN_POINT ( 'NONE',  ( -70.18950016389896973, -196.7549604899246560, -360.5100559345433453 ) ) ;
#84817=CARTESIAN_POINT ( 'NONE',  ( -35.36684806826554706, -276.0771255001219515, -195.5410233525968522 ) ) ;
#84818=CARTESIAN_POINT ( 'NONE',  ( -22.85399180902964744, -107.9061763485807575, -362.3883434141006319 ) ) ;
#84819=CARTESIAN_POINT ( 'NONE',  ( -38.35132707659149531, -278.0595478403196807, -195.7104624054299222 ) ) ;
#84820=CARTESIAN_POINT ( 'NONE',  ( 3.576728897784181793, -294.3541604621228771, -206.2702029395413774 ) ) ;
#84821=CARTESIAN_POINT ( 'NONE',  ( -106.0858749912648165, -295.5682328616630912, -295.3722504882852604 ) ) ;
#84822=CARTESIAN_POINT ( 'NONE',  ( -114.3071169708805002, -290.0849770803972092, -268.3500589904878666 ) ) ;
#84824=CARTESIAN_POINT ( 'NONE',  ( -65.40412269765339204, -293.9866170260205536, -341.4463711949826461 ) ) ;
#84825=CARTESIAN_POINT ( 'NONE',  ( -7.917463025506221719, -284.8441096491782218, -202.6805839453087685 ) ) ;
#84826=CARTESIAN_POINT ( 'NONE',  ( -22.51672697835618564, -294.1043819849616625, -197.6212688720690096 ) ) ;
#84827=CARTESIAN_POINT ( 'NONE',  ( -6.710822767611735351, -284.9416101420918608, -203.3214644756497762 ) ) ;
#84828=CARTESIAN_POINT ( 'NONE',  ( -110.8110360097829954, -285.8238852202031808, -273.6769757991029337 ) ) ;
#84830=CARTESIAN_POINT ( 'NONE',  ( -110.2113524460009444, -291.8000903049033923, -246.0527354650368750 ) ) ;
#84831=CARTESIAN_POINT ( 'NONE',  ( -40.23052004740426923, -283.5817903235462154, -343.3655230638606781 ) ) ;
#84832=CARTESIAN_POINT ( 'NONE',  ( -90.44791490317665250, -294.5786128598911091, -325.6404907111116245 ) ) ;
#84833=CARTESIAN_POINT ( 'NONE',  ( -112.1031967444912425, -291.1318852902273875, -288.1621713047666731 ) ) ;
#84834=CARTESIAN_POINT ( 'NONE',  ( -113.7516712763731590, -290.9263203072271722, -279.8029483380072406 ) ) ;
#84835=CARTESIAN_POINT ( 'NONE',  ( 33.70157724005862576, -287.9403130411283200, -287.1495885898339111 ) ) ;
#84838=CARTESIAN_POINT ( 'NONE',  ( -55.74692182794782269, -297.1470581060739278, -343.8563783195525048 ) ) ;
#84839=CARTESIAN_POINT ( 'NONE',  ( -67.96458247795152374, -296.3434408782087530, -200.1937976084643367 ) ) ;
#84840=CARTESIAN_POINT ( 'NONE',  ( -74.61525198448114793, -278.6021579599489542, -207.2624438366001698 ) ) ;
#84841=ORIENTED_EDGE ( 'NONE', *, *, #72825, .F. ) ;
#84842=CARTESIAN_POINT ( 'NONE',  ( 39.07569942218166403, -275.1772789667185179, -279.7466177749163307 ) ) ;
#84843=CARTESIAN_POINT ( 'NONE',  ( -75.55375752995296068, -296.0126425416032134, -207.2896907608808590 ) ) ;
#84844=CARTESIAN_POINT ( 'NONE',  ( 12.59584276663795066, -278.2080731425076010, -325.3590930503311824 ) ) ;
#84845=CARTESIAN_POINT ( 'NONE',  ( -2.310188958453692987, -272.6605247745145562, -204.9114525339362274 ) ) ;
#84846=CARTESIAN_POINT ( 'NONE',  ( -41.04398173148692308, -296.3048248823506583, -343.6773935663883321 ) ) ;
#84847=CARTESIAN_POINT ( 'NONE',  ( -26.14669701250242895, -295.9859452670694964, -342.8103966413188459 ) ) ;
#84849=CARTESIAN_POINT ( 'NONE',  ( -34.86007271588531609, -296.6215858104486074, -346.5207000627032130 ) ) ;
#84850=CARTESIAN_POINT ( 'NONE',  ( -69.91106507176493778, -295.6240379100742075, -202.6170045935101029 ) ) ;
#84851=CARTESIAN_POINT ( 'NONE',  ( -57.69126134834083786, -292.4339055353319168, -200.0957162742227240 ) ) ;
#84852=CARTESIAN_POINT ( 'NONE',  ( -83.49128943082487808, -274.2405127590476468, -208.8585822593338150 ) ) ;
#84853=CARTESIAN_POINT ( 'NONE',  ( -108.2987918063060135, -288.8689973908423667, -290.0546149252017472 ) ) ;
#84854=CARTESIAN_POINT ( 'NONE',  ( 72.69263585473569833, -301.4297953448794374, -195.3235991646452305 ) ) ;
#84855=CARTESIAN_POINT ( 'NONE',  ( -99.52102728028046386, -273.6473780954311792, -224.9598749675746490 ) ) ;
#84856=CARTESIAN_POINT ( 'NONE',  ( -65.58481138269844735, -298.0056301264149283, -203.0230592528929776 ) ) ;
#84857=CARTESIAN_POINT ( 'NONE',  ( -1.931131629580074893, -282.4987032624279664, -203.8442145391391875 ) ) ;
#84858=CARTESIAN_POINT ( 'NONE',  ( 12.68245189519852190, -279.4178322048057908, -212.4743104539741125 ) ) ;
#84859=CARTESIAN_POINT ( 'NONE',  ( -107.4865335111504834, -277.4962938740018785, -302.0028618746571283 ) ) ;
#84861=CARTESIAN_POINT ( 'NONE',  ( -17.18380655957072278, -278.7080205149388235, -196.8757470545449451 ) ) ;
#84862=CARTESIAN_POINT ( 'NONE',  ( 31.86769885117764289, -279.9358960448640801, -299.8211820090648985 ) ) ;
#84863=CARTESIAN_POINT ( 'NONE',  ( -54.33008881778547305, -272.4043472460634234, -198.7596545537465715 ) ) ;
#84864=CARTESIAN_POINT ( 'NONE',  ( -5.607782151842636509, -278.6350174575242704, -338.3305266278346153 ) ) ;
#84867=CARTESIAN_POINT ( 'NONE',  ( -65.15000598038282931, -295.9337240579027366, -199.5894554512790364 ) ) ;
#84869=CARTESIAN_POINT ( 'NONE',  ( -37.79503013874025896, -292.0466210835031120, -193.3624524622963747 ) ) ;
#84870=CARTESIAN_POINT ( 'NONE',  ( 32.49071750981946849, -277.9153491248761156, -298.3127502029152538 ) ) ;
#84871=CARTESIAN_POINT ( 'NONE',  ( -8.170028999098940758, -272.4338772151675698, -201.2114776745634117 ) ) ;
#84872=DIRECTION ( 'NONE',  ( 1.000000000000000000, 0.000000000000000000, 0.000000000000000000 ) ) ;
#84873=CARTESIAN_POINT ( 'NONE',  ( -49.83095356496649231, -285.1302866145171038, -344.9346702000764253 ) ) ;
#84875=CARTESIAN_POINT ( 'NONE',  ( -1.551112478440801468, -284.5260410164028144, -204.3946948250082869 ) ) ;
#84877=CARTESIAN_POINT ( 'NONE',  ( 18.26326524469824619, -293.0258933389397953, -318.2887129829994137 ) ) ;
#84878=CARTESIAN_POINT ( 'NONE',  ( 36.18046615318034753, -285.8260804812475158, -280.7177935575422225 ) ) ;
#84880=CARTESIAN_POINT ( 'NONE',  ( 11.57728245303386316, -292.3731666270389837, -327.2112172708158937 ) ) ;
#84881=CARTESIAN_POINT ( 'NONE',  ( -23.88894097986979759, -284.7007541918591755, -195.1959296855863215 ) ) ;
#84882=CARTESIAN_POINT ( 'NONE',  ( -111.1924062690921176, -280.1483698570180536, -270.6614252967327161 ) ) ;
#84883=CARTESIAN_POINT ( 'NONE',  ( -4.955841750281797964, -287.6742364407118657, -200.9409127292508686 ) ) ;
#84884=CARTESIAN_POINT ( 'NONE',  ( 29.83657330895386295, -279.3260770113772082, -234.7375636802884742 ) ) ;
#84885=CARTESIAN_POINT ( 'NONE',  ( 35.27439374902280633, -287.4535204284661631, -262.8842931195853794 ) ) ;
#84886=CARTESIAN_POINT ( 'NONE',  ( -27.49737763341369501, -281.6048002811040760, -197.3817137364107737 ) ) ;
#84887=CARTESIAN_POINT ( 'NONE',  ( -51.86940424075815059, -280.6644473029521123, -198.6046865971727300 ) ) ;
#84889=CARTESIAN_POINT ( 'NONE',  ( -29.65630261754789032, -288.1289141567871752, -195.3988510269741710 ) ) ;
#84891=CARTESIAN_POINT ( 'NONE',  ( -91.63402372937669327, -297.1375136660911380, -215.7594366671517037 ) ) ;
#84892=CARTESIAN_POINT ( 'NONE',  ( -81.35751155469240814, -291.6334289761899754, -330.7118640853988154 ) ) ;
#84894=CARTESIAN_POINT ( 'NONE',  ( -54.49178911615187815, -276.3376638359844151, -195.3683826091709363 ) ) ;
#84896=CARTESIAN_POINT ( 'NONE',  ( -84.63452168851617330, -271.4021107462828581, -211.9366586157784695 ) ) ;
#84899=CARTESIAN_POINT ( 'NONE',  ( -41.91809878868544104, -293.5086537330012675, -346.4754211083483142 ) ) ;
#84900=CARTESIAN_POINT ( 'NONE',  ( -39.16358283339859270, -297.5363618254613698, -197.3098788183234547 ) ) ;
#84901=CARTESIAN_POINT ( 'NONE',  ( -23.63743177913956117, -290.3941044910961295, -342.8211883146426544 ) ) ;
#84902=CARTESIAN_POINT ( 'NONE',  ( 29.88382654553237927, -282.8988336313091736, -239.2754536350166745 ) ) ;
#84903=CARTESIAN_POINT ( 'NONE',  ( -36.07824168314350999, -290.4619016368691291, -346.7744547805619959 ) ) ;
#84904=CARTESIAN_POINT ( 'NONE',  ( -57.14698346822036967, -290.6175147624210808, -344.3147773715898552 ) ) ;
#84905=CARTESIAN_POINT ( 'NONE',  ( -70.89955365870332571, -287.6096530891726957, -203.2731652206429942 ) ) ;
#84906=CARTESIAN_POINT ( 'NONE',  ( -67.36441661612408893, -279.8358102449926719, -199.4552895959129728 ) ) ;
#84907=CARTESIAN_POINT ( 'NONE',  ( -58.47250858125631368, -293.4029460493510442, -342.9608360133648830 ) ) ;
#84908=CARTESIAN_POINT ( 'NONE',  ( 35.60840098083281191, -281.6977358413952288, -295.1699114067511687 ) ) ;
#84909=CARTESIAN_POINT ( 'NONE',  ( 36.83746114244013370, -277.4643956643378715, -274.3558725303914230 ) ) ;
#84911=CARTESIAN_POINT ( 'NONE',  ( 17.40634833298267736, -278.6948066931273047, -313.9805196606274080 ) ) ;
#84912=CARTESIAN_POINT ( 'NONE',  ( 31.64265073936129724, -273.3775357678563296, -238.3745803437362838 ) ) ;
#84913=CARTESIAN_POINT ( 'NONE',  ( 19.39586235373092649, -281.7107656293368336, -316.4116675856188863 ) ) ;
#84914=CARTESIAN_POINT ( 'NONE',  ( -75.12691378274729459, -278.7491654808909516, -336.9965916272910817 ) ) ;
#84915=CARTESIAN_POINT ( 'NONE',  ( -104.8392231956981817, -274.2569284932557707, -241.1575596628881613 ) ) ;
#84916=CARTESIAN_POINT ( 'NONE',  ( -112.7647670213274154, -283.7935797413243790, -255.7955779959871734 ) ) ;
#84917=CARTESIAN_POINT ( 'NONE',  ( -109.0963412854132031, -292.5491035610610879, -252.1643872380254265 ) ) ;
#84918=CARTESIAN_POINT ( 'NONE',  ( -68.53540802779889418, -275.2492049255736788, -200.8242624724241523 ) ) ;
#84919=CARTESIAN_POINT ( 'NONE',  ( -105.1794743133070256, -274.3278742879541028, -234.8723594374499442 ) ) ;
#84921=CARTESIAN_POINT ( 'NONE',  ( -19.01899488175570951, -276.6429645257778134, -341.0242517719701141 ) ) ;
#84922=CARTESIAN_POINT ( 'NONE',  ( -111.9241880270047602, -298.4657364798912909, -277.0891985200167937 ) ) ;
#84923=CARTESIAN_POINT ( 'NONE',  ( -68.28304432140735969, -283.6446333453809530, -202.2240381397060673 ) ) ;
#84924=CARTESIAN_POINT ( 'NONE',  ( -0.8101501031219983107, -292.1905315015141582, -202.6027963951183608 ) ) ;
#84925=CARTESIAN_POINT ( 'NONE',  ( 25.18474047723890052, -273.0197794820817876, -229.5899145719604348 ) ) ;
#84926=CARTESIAN_POINT ( 'NONE',  ( 38.80595800771392589, -289.2028216164353012, -274.3604172580151044 ) ) ;
#84927=CARTESIAN_POINT ( 'NONE',  ( -103.1288549890172277, -289.0360352589741524, -302.7073129355213723 ) ) ;
#84929=CARTESIAN_POINT ( 'NONE',  ( -73.14146154720549475, -290.1618383140167339, -202.8409016208236437 ) ) ;
#84930=CARTESIAN_POINT ( 'NONE',  ( -96.77609858494014361, -290.8124272117787541, -227.8534361110645250 ) ) ;
#84932=CARTESIAN_POINT ( 'NONE',  ( 38.24983755128842233, -288.4683809945918256, -257.3451653380889752 ) ) ;
#84933=CARTESIAN_POINT ( 'NONE',  ( -110.4130751150576515, -278.8817264824106132, -270.6423695624922630 ) ) ;
#84934=CARTESIAN_POINT ( 'NONE',  ( -19.37310057854351797, -293.7466992563412305, -344.9719473593676184 ) ) ;
#84935=CARTESIAN_POINT ( 'NONE',  ( -37.98991983772272363, -286.6956400288447639, -193.4657826341520206 ) ) ;
#84936=CARTESIAN_POINT ( 'NONE',  ( -87.73930435206074208, -285.7040590267891389, -212.1026971947967752 ) ) ;
#84937=CARTESIAN_POINT ( 'NONE',  ( 32.25276550568090528, -282.1804106144927573, -292.6323394454112758 ) ) ;
#84938=CARTESIAN_POINT ( 'NONE',  ( 153.9038455766559252, 207.1106375885822786, -217.3830698506460521 ) ) ;
#84940=CARTESIAN_POINT ( 'NONE',  ( 166.5459560125245275, 232.5563224728020373, -191.9177544221001028 ) ) ;
#84941=CARTESIAN_POINT ( 'NONE',  ( 192.2295762369160457, 276.4233758247025889, -124.0683339759032435 ) ) ;
#84943=CARTESIAN_POINT ( 'NONE',  ( 17.41319056084516959, -274.0568178855980932, -221.7628093281351482 ) ) ;
#84944=CARTESIAN_POINT ( 'NONE',  ( 33.16109047770582663, -274.2058278414356209, -250.0902415138952506 ) ) ;
#84945=CARTESIAN_POINT ( 'NONE',  ( -114.3048253765348647, -296.0335123176099614, -272.4618511282888562 ) ) ;
#84946=CARTESIAN_POINT ( 'NONE',  ( 26.53395668783571182, -24.55290782687918139, -341.8058727006235813 ) ) ;
#84947=CARTESIAN_POINT ( 'NONE',  ( 23.96239827260135868, -274.8498358534708927, -316.1334436095236811 ) ) ;
#84948=CARTESIAN_POINT ( 'NONE',  ( -89.00205447178591101, -299.1775367070667926, -216.9782278248142404 ) ) ;
#84949=CARTESIAN_POINT ( 'NONE',  ( -81.92789847499841471, -292.5081938149662051, -212.1049742978525785 ) ) ;
#84951=CARTESIAN_POINT ( 'NONE',  ( -110.9862564060357073, -297.2203015256591243, -292.0707797470780065 ) ) ;
#84953=CARTESIAN_POINT ( 'NONE',  ( 34.58337333767331501, -288.2136916304594365, -283.1974822935964653 ) ) ;
#84954=CARTESIAN_POINT ( 'NONE',  ( -112.4451590605510063, -297.1514918223394943, -286.5977825920128907 ) ) ;
#84955=CARTESIAN_POINT ( 'NONE',  ( -58.82811829318622188, -295.8150589477813810, -344.2939800234042877 ) ) ;
#84956=CARTESIAN_POINT ( 'NONE',  ( 16.73675102980893570, -293.0155130479860190, -221.2510649776955063 ) ) ;
#84958=CARTESIAN_POINT ( 'NONE',  ( 35.11960803832374012, -277.7466278287836303, -291.8234714321406500 ) ) ;
#84960=CARTESIAN_POINT ( 'NONE',  ( -8.878044875214289533, -279.9223401578673247, -198.8814199354349057 ) ) ;
#84961=CARTESIAN_POINT ( 'NONE',  ( 13.90451201885680987, -277.2532243289963958, -322.7503405305836282 ) ) ;
#84962=CARTESIAN_POINT ( 'NONE',  ( 36.94986507705546330, -277.1092387535302350, -254.3391954089093190 ) ) ;
#84963=CARTESIAN_POINT ( 'NONE',  ( -111.1869626077413642, -276.3796360804223582, -285.4344538218659864 ) ) ;
#84964=CARTESIAN_POINT ( 'NONE',  ( -103.8147315674224984, -297.6146669658842256, -239.8216752366159028 ) ) ;
#84965=CARTESIAN_POINT ( 'NONE',  ( -67.55358021487614906, -294.0311696544250140, -337.4764806566925017 ) ) ;
#84966=CARTESIAN_POINT ( 'NONE',  ( -107.5173985441935969, -278.6398702184750391, -302.0327398168233799 ) ) ;
#84967=CARTESIAN_POINT ( 'NONE',  ( -68.03548982078876861, -277.6334048858773826, -336.6084767317124147 ) ) ;
#84970=CARTESIAN_POINT ( 'NONE',  ( 32.27032689822701172, -285.8271789734006916, -238.4929518292211412 ) ) ;
#84971=CARTESIAN_POINT ( 'NONE',  ( -23.79882560928694701, -300.2214628073405720, -195.1898382442023774 ) ) ;
#84972=CARTESIAN_POINT ( 'NONE',  ( 82.63422563859604963, -300.7068507995575715, -197.5857633699117741 ) ) ;
#84973=CARTESIAN_POINT ( 'NONE',  ( 34.16633119161235044, -286.9536168546941894, -285.8860302165797407 ) ) ;
#84974=CARTESIAN_POINT ( 'NONE',  ( -52.00651184383531955, -278.1018859024631524, -197.7627052112191564 ) ) ;
#84975=CARTESIAN_POINT ( 'NONE',  ( -38.34378613340424380, -278.6140778668016651, -196.7662097404028998 ) ) ;
#84976=CARTESIAN_POINT ( 'NONE',  ( -109.1567198465016730, -282.3775832054524813, -290.0031066220593630 ) ) ;
#84977=CARTESIAN_POINT ( 'NONE',  ( -37.40560091916179886, -288.0514730517481894, -195.3485665393942554 ) ) ;
#84978=CARTESIAN_POINT ( 'NONE',  ( 21.16266784627691067, -277.3766754572978925, -314.6823254777914372 ) ) ;
#84980=CARTESIAN_POINT ( 'NONE',  ( -91.38897937504209779, -293.2837682531524024, -218.2882407209644953 ) ) ;
#84981=CARTESIAN_POINT ( 'NONE',  ( -110.4714660641430015, -276.5298901964705465, -291.0011603537972178 ) ) ;
#84982=CARTESIAN_POINT ( 'NONE',  ( -9.942470107421407022, -277.3360991616660272, -338.1476689253897803 ) ) ;
#84983=CARTESIAN_POINT ( 'NONE',  ( 21.11399038967085318, -284.2015567204788908, -317.6356483939983377 ) ) ;
#84985=CARTESIAN_POINT ( 'NONE',  ( 35.97356913955299973, -289.2392332292763513, -252.0803769219947981 ) ) ;
#84986=CARTESIAN_POINT ( 'NONE',  ( -100.8917166006252444, -295.0883993059197223, -230.4351542719718395 ) ) ;
#84988=CARTESIAN_POINT ( 'NONE',  ( -36.71515387767735916, -272.7450092991016959, -196.8581369266514685 ) ) ;
#84989=CARTESIAN_POINT ( 'NONE',  ( 35.16122893312238062, -291.4841527466867888, -254.3588944933474636 ) ) ;
#84992=CARTESIAN_POINT ( 'NONE',  ( -39.17545016596928065, -290.5094486551427053, -194.0635676381172914 ) ) ;
#84993=CARTESIAN_POINT ( 'NONE',  ( -109.1996264325236581, -285.9321616995211457, -287.2352679458221587 ) ) ;
#84994=CARTESIAN_POINT ( 'NONE',  ( 38.56668245091941571, -285.7354812931919241, -265.9005228054472241 ) ) ;
#84995=CARTESIAN_POINT ( 'NONE',  ( -106.7232414177929058, -285.6518306470258040, -295.0398112443616583 ) ) ;
#84996=CARTESIAN_POINT ( 'NONE',  ( -62.62825852687898021, -286.5174504684008525, -201.6543986694567536 ) ) ;
#84998=CARTESIAN_POINT ( 'NONE',  ( -33.64580452643579633, -294.0783471029640168, -195.0966033673003608 ) ) ;
#84999=CARTESIAN_POINT ( 'NONE',  ( 27.84113642410498812, -274.1389517394873678, -308.5777637675636811 ) ) ;
#85001=CARTESIAN_POINT ( 'NONE',  ( 36.86637103746694777, -276.1424552926130218, -290.8774825076309298 ) ) ;
#85003=CARTESIAN_POINT ( 'NONE',  ( -103.3400973420037019, -289.1180632144612446, -233.5708235992334778 ) ) ;
#85004=CARTESIAN_POINT ( 'NONE',  ( -97.92890798767126626, -277.9168926245682201, -317.8815372123905263 ) ) ;
#85005=CARTESIAN_POINT ( 'NONE',  ( -108.4280933938048719, -298.2347514992417814, -293.3004310822690854 ) ) ;
#85008=CARTESIAN_POINT ( 'NONE',  ( -107.8231473814541062, -283.5127527382658741, -249.3614744254330446 ) ) ;
#85010=CARTESIAN_POINT ( 'NONE',  ( -47.81366247784037427, -277.9189514113317045, -196.0433481135916622 ) ) ;
#85012=CARTESIAN_POINT ( 'NONE',  ( 29.35105616525251548, -273.5458214539480082, -233.1743350792007732 ) ) ;
#85013=CARTESIAN_POINT ( 'NONE',  ( -108.5874797671769869, -277.6843782749242564, -286.7852344899939112 ) ) ;
#85015=CARTESIAN_POINT ( 'NONE',  ( 17.61037683689601607, -295.7682070007553534, -319.4818498119317951 ) ) ;
#85016=CARTESIAN_POINT ( 'NONE',  ( 34.04176770134874630, -280.1140271836077886, -242.1823243726990711 ) ) ;
#85017=CARTESIAN_POINT ( 'NONE',  ( -78.07067670734340936, -296.5554807102024029, -331.2874521303659208 ) ) ;
#85018=CARTESIAN_POINT ( 'NONE',  ( -3.432195700594277810, -295.9290958468386634, -338.9572874588480431 ) ) ;
#85019=CARTESIAN_POINT ( 'NONE',  ( -94.44999314464222095, -297.0276148570155215, -224.8897767523308175 ) ) ;
#85020=CARTESIAN_POINT ( 'NONE',  ( -14.25428822253264727, -294.3517285943561319, -199.0030626670235279 ) ) ;
#85021=CARTESIAN_POINT ( 'NONE',  ( -32.30853939835375144, -286.2806215865667809, -193.5126258549709632 ) ) ;
#85022=CARTESIAN_POINT ( 'NONE',  ( 23.50230962071297469, -273.0816993731379512, -225.2134495984524278 ) ) ;
#85023=CARTESIAN_POINT ( 'NONE',  ( 3.178330159813210987, -288.3574600643131589, -335.8998220271025730 ) ) ;
#85024=CARTESIAN_POINT ( 'NONE',  ( -34.27033393422726704, -282.0708196800877090, -195.7667020218742664 ) ) ;
#85026=CARTESIAN_POINT ( 'NONE',  ( -14.48121458390158089, -285.4145089231023462, -200.7320195045245441 ) ) ;
#85027=CARTESIAN_POINT ( 'NONE',  ( -88.15564890472626303, -287.7633390326610083, -325.5239973142273584 ) ) ;
#85028=CARTESIAN_POINT ( 'NONE',  ( -98.31850732666445936, -258.1384851437703674, -325.6453615436536211 ) ) ;
#85029=CARTESIAN_POINT ( 'NONE',  ( 26.42414952981355469, -286.5711500632839943, -234.5938157740320378 ) ) ;
#85031=CARTESIAN_POINT ( 'NONE',  ( 24.92348424847820354, -283.0907775280153942, -315.2818436728126130 ) ) ;
#85033=CARTESIAN_POINT ( 'NONE',  ( -103.0083337835546047, -290.1325745038440687, -230.5004701966750531 ) ) ;
#85034=CARTESIAN_POINT ( 'NONE',  ( -95.31061226682197685, -280.8265108970002757, -220.8835565826972527 ) ) ;
#85035=CARTESIAN_POINT ( 'NONE',  ( -92.72838467810875329, -280.5942064235289308, -217.5064947537138949 ) ) ;
#85036=CARTESIAN_POINT ( 'NONE',  ( 32.23067187854067583, -281.6805300397424503, -292.6319561521697210 ) ) ;
#85037=CARTESIAN_POINT ( 'NONE',  ( 34.43772122113939105, -277.8330348420646487, -292.1477060132437487 ) ) ;
#85038=CARTESIAN_POINT ( 'NONE',  ( 24.88627965927573626, -294.1543096074584014, -315.7339456628644712 ) ) ;
#85039=CARTESIAN_POINT ( 'NONE',  ( -110.0233630504302909, -288.7923819366740190, -253.2989071530174954 ) ) ;
#85041=CARTESIAN_POINT ( 'NONE',  ( -110.5510762278442201, -295.4222589701827246, -274.1838557289810296 ) ) ;
#85044=CARTESIAN_POINT ( 'NONE',  ( 35.35181989373702294, -283.6796792428266372, -286.3912879321316041 ) ) ;
#85045=CARTESIAN_POINT ( 'NONE',  ( -84.49499115023635909, -295.3889148290286357, -326.1828206211164343 ) ) ;
#85046=( BOUNDED_SURFACE ( )  B_SPLINE_SURFACE ( 3, 3, ( 
 ( #41429, #18748, #70816, #57545, #79773, #71765, #51340, #13066, #13988, #71284, #27729, #41902, #64214, #42849, #78842, #79329, #93043, #6888, #22022, #86390, #50424, #63733, #236, #43771 ),
 ( #5948, #34820, #21541, #14916, #35762, #92558, #56626, #64675, #6411, #85476, #20623, #28200, #93502, #28657, #14466, #57088, #43323, #50892, #72219, #7335, #49494, #29116, #72672, #78383 ),
 ( #13524, #7792, #58012, #712, #35286, #42372, #85928, #29597, #36215, #21078, #36677, #65599, #49949, #65135, #86868, #87320, #58476, #22468, #73605, #81158, #73141, #24805, #67441, #2099 ),
 ( #1623, #16763, #52731, #74054, #1167, #59401, #81614, #15370, #60336, #23865, #9173, #51801, #8267, #87781, #16302, #30506, #30990, #58931, #88255, #44704, #45617, #2568, #89635, #75005 ),
 ( #45155, #15847, #74518, #88717, #37147, #52279, #89173, #9653, #80693, #38538, #22931, #3019, #23413, #31447, #66960, #53202, #66504, #30050, #38983, #24325, #44232, #80234, #59877, #8716 ),
 ( #37593, #38051, #82080, #66054, #17238, #46100, #10117, #67896, #60797, #31905, #83473, #26675, #69758, #68358, #11526, #19561, #11990, #39442, #46559, #32838, #84413, #4419, #10579, #17706 ),
 ( #19106, #48427, #47961, #47495, #70249, #54143, #83012, #62195, #3486, #54602, #18164, #76865, #91025, #75458, #25718, #33773, #26194, #47017, #55088, #90114, #5384, #61728, #40839, #40373 ) ),
 .UNSPECIFIED., .T., .F., .F. ) 
 B_SPLINE_SURFACE_WITH_KNOTS ( ( 4, 3, 4 ),
 ( 4, 2, 2, 2, 2, 2, 2, 2, 2, 2, 2, 4 ),
 ( 0.000000000000000000, 0.5000000000000000000, 1.000000000000000000 ),
 ( 0.000000000000000000, 0.06250000000000000000, 0.1250000000000000000, 0.2500000000000000000, 0.3750000000000000000, 0.5000000000000000000, 0.6250000000000000000, 0.7500000000000000000, 0.8125000000000000000, 0.8750000000000000000, 0.9375000000000000000, 1.000000000000000000 ),
 .UNSPECIFIED. ) 
 GEOMETRIC_REPRESENTATION_ITEM ( )  RATIONAL_B_SPLINE_SURFACE ( (
 ( 1.000000000000000000, 1.000000000000000000, 1.000000000000000000, 1.000000000000000000, 1.000000000000000000, 1.000000000000000000, 1.000000000000000000, 1.000000000000000000, 1.000000000000000000, 1.000000000000000000, 1.000000000000000000, 1.000000000000000000, 1.000000000000000000, 1.000000000000000000, 1.000000000000000000, 1.000000000000000000, 1.000000000000000000, 1.000000000000000000, 1.000000000000000000, 1.000000000000000000, 1.000000000000000000, 1.000000000000000000, 1.000000000000000000, 1.000000000000000000),
 ( 0.3333333333333333703, 0.3333333333333333703, 0.3333333333333333703, 0.3333333333333333703, 0.3333333333333333703, 0.3333333333333333703, 0.3333333333333333703, 0.3333333333333333703, 0.3333333333333333703, 0.3333333333333333703, 0.3333333333333333703, 0.3333333333333333703, 0.3333333333333333703, 0.3333333333333333703, 0.3333333333333333703, 0.3333333333333333703, 0.3333333333333333703, 0.3333333333333333703, 0.3333333333333333703, 0.3333333333333333703, 0.3333333333333333703, 0.3333333333333333703, 0.3333333333333333703, 0.3333333333333333703),
 ( 0.3333333333333333703, 0.3333333333333333703, 0.3333333333333333703, 0.3333333333333333703, 0.3333333333333333703, 0.3333333333333333703, 0.3333333333333333703, 0.3333333333333333703, 0.3333333333333333703, 0.3333333333333333703, 0.3333333333333333703, 0.3333333333333333703, 0.3333333333333333703, 0.3333333333333333703, 0.3333333333333333703, 0.3333333333333333703, 0.3333333333333333703, 0.3333333333333333703, 0.3333333333333333703, 0.3333333333333333703, 0.3333333333333333703, 0.3333333333333333703, 0.3333333333333333703, 0.3333333333333333703),
 ( 1.000000000000000000, 1.000000000000000000, 1.000000000000000000, 1.000000000000000000, 1.000000000000000000, 1.000000000000000000, 1.000000000000000000, 1.000000000000000000, 1.000000000000000000, 1.000000000000000000, 1.000000000000000000, 1.000000000000000000, 1.000000000000000000, 1.000000000000000000, 1.000000000000000000, 1.000000000000000000, 1.000000000000000000, 1.000000000000000000, 1.000000000000000000, 1.000000000000000000, 1.000000000000000000, 1.000000000000000000, 1.000000000000000000, 1.000000000000000000),
 ( 0.3333333333333333703, 0.3333333333333333703, 0.3333333333333333703, 0.3333333333333333703, 0.3333333333333333703, 0.3333333333333333703, 0.3333333333333333703, 0.3333333333333333703, 0.3333333333333333703, 0.3333333333333333703, 0.3333333333333333703, 0.3333333333333333703, 0.3333333333333333703, 0.3333333333333333703, 0.3333333333333333703, 0.3333333333333333703, 0.3333333333333333703, 0.3333333333333333703, 0.3333333333333333703, 0.3333333333333333703, 0.3333333333333333703, 0.3333333333333333703, 0.3333333333333333703, 0.3333333333333333703),
 ( 0.3333333333333333703, 0.3333333333333333703, 0.3333333333333333703, 0.3333333333333333703, 0.3333333333333333703, 0.3333333333333333703, 0.3333333333333333703, 0.3333333333333333703, 0.3333333333333333703, 0.3333333333333333703, 0.3333333333333333703, 0.3333333333333333703, 0.3333333333333333703, 0.3333333333333333703, 0.3333333333333333703, 0.3333333333333333703, 0.3333333333333333703, 0.3333333333333333703, 0.3333333333333333703, 0.3333333333333333703, 0.3333333333333333703, 0.3333333333333333703, 0.3333333333333333703, 0.3333333333333333703),
 ( 1.000000000000000000, 1.000000000000000000, 1.000000000000000000, 1.000000000000000000, 1.000000000000000000, 1.000000000000000000, 1.000000000000000000, 1.000000000000000000, 1.000000000000000000, 1.000000000000000000, 1.000000000000000000, 1.000000000000000000, 1.000000000000000000, 1.000000000000000000, 1.000000000000000000, 1.000000000000000000, 1.000000000000000000, 1.000000000000000000, 1.000000000000000000, 1.000000000000000000, 1.000000000000000000, 1.000000000000000000, 1.000000000000000000, 1.000000000000000000) ) ) 
 REPRESENTATION_ITEM ( '' )  SURFACE ( )  );
#85047=CARTESIAN_POINT ( 'NONE',  ( 37.11851156330262569, -294.4011836843862966, -251.9989452932912570 ) ) ;
#85048=CARTESIAN_POINT ( 'NONE',  ( -61.56067988772937127, -284.0265586835061526, -339.3878532841630999 ) ) ;
#85049=CARTESIAN_POINT ( 'NONE',  ( -34.10109514277978349, -273.1507284015519872, -193.6648423704500033 ) ) ;
#85050=CARTESIAN_POINT ( 'NONE',  ( -113.2580984399872790, -291.0501817850090447, -282.6091077774356108 ) ) ;
#85051=CARTESIAN_POINT ( 'NONE',  ( -26.76964319381484358, -284.3246883260927689, -195.2848990172662695 ) ) ;
#85052=CARTESIAN_POINT ( 'NONE',  ( -113.9862107040246570, -290.9819809125345955, -262.6433005713994930 ) ) ;
#85053=CARTESIAN_POINT ( 'NONE',  ( -21.12051624089891888, -289.1715224738794632, -341.5577518915829955 ) ) ;
#85056=CARTESIAN_POINT ( 'NONE',  ( 188.8180124195482108, 268.1546957682879224, -137.4927483566484341 ) ) ;
#85057=CARTESIAN_POINT ( 'NONE',  ( -0.6912889005501295925, -284.0945348494694258, -337.3046558309981151 ) ) ;
#85058=CARTESIAN_POINT ( 'NONE',  ( 10.59707575819633618, -279.9094976428775681, -330.5268031993606428 ) ) ;
#85059=ORIENTED_EDGE ( 'NONE', *, *, #13462, .T. ) ;
#85060=CARTESIAN_POINT ( 'NONE',  ( 7.974294312517242744, -281.3367078454543844, -328.0513402115038275 ) ) ;
#85061=CARTESIAN_POINT ( 'NONE',  ( 1.032808759574668445, -276.2216535144020781, -337.1534396982845010 ) ) ;
#85062=CARTESIAN_POINT ( 'NONE',  ( -77.31410124693465491, -279.5892618874532900, -333.6852744555749837 ) ) ;
#85063=CARTESIAN_POINT ( 'NONE',  ( 175.1846718914974588, 240.5146751456763923, -177.8570858195099333 ) ) ;
#85064=CARTESIAN_POINT ( 'NONE',  ( 30.20946171836731153, -279.6608920481897371, -234.5348671969436793 ) ) ;
#85065=CARTESIAN_POINT ( 'NONE',  ( -49.66887700636713276, -283.9144179399754080, -196.6885766365219297 ) ) ;
#85066=CARTESIAN_POINT ( 'NONE',  ( -97.44640746834767242, -298.9414116627343105, -223.8492702237638241 ) ) ;
#85067=CARTESIAN_POINT ( 'NONE',  ( 35.35589676719921215, -293.9420632498192276, -262.5891425576214715 ) ) ;
#85069=CARTESIAN_POINT ( 'NONE',  ( -98.70210651318809880, -289.7953113110343111, -229.8194318841307791 ) ) ;
#85070=CARTESIAN_POINT ( 'NONE',  ( 37.18438702983876709, -275.9660981556214665, -251.4092019869858063 ) ) ;
#85071=CARTESIAN_POINT ( 'NONE',  ( -103.2050763408169303, -272.9778981233729951, -238.8807165578695049 ) ) ;
#85073=CARTESIAN_POINT ( 'NONE',  ( -55.24805428201199220, -272.7473504839670113, -195.7899775206671791 ) ) ;
#85079=CARTESIAN_POINT ( 'NONE',  ( 7.995872605634569474, -283.4957032231836820, -328.0343832530571717 ) ) ;
#85080=CARTESIAN_POINT ( 'NONE',  ( -39.58016678030841717, -281.7845742691787336, -194.3945476324544757 ) ) ;
#85081=CARTESIAN_POINT ( 'NONE',  ( -59.02920927561647346, -282.3983754484648898, -340.3648477261895664 ) ) ;
#85082=CARTESIAN_POINT ( 'NONE',  ( 36.80074759569227894, -283.4606995728644847, -274.0709594013600281 ) ) ;
#85083=CARTESIAN_POINT ( 'NONE',  ( 36.39223134863493669, -274.0484193847123038, -271.6159080386087794 ) ) ;
#85087=AXIS2_PLACEMENT_3D ( 'NONE', #25915, #54798, #47695 ) ;
#85088=CARTESIAN_POINT ( 'NONE',  ( -65.02732640655588625, -278.2074936529761544, -342.0947888608088192 ) ) ;
#85092=CARTESIAN_POINT ( 'NONE',  ( -96.73218599766430259, -285.8987548337361204, -316.7419005904325218 ) ) ;
#85094=CARTESIAN_POINT ( 'NONE',  ( -5.963122567394080420, -291.6726536459932504, -204.2565593400196349 ) ) ;
#85095=CARTESIAN_POINT ( 'NONE',  ( -38.92640092054078593, -288.4201354131334369, -347.2428551534226813 ) ) ;
#85096=CARTESIAN_POINT ( 'NONE',  ( -49.56713993043211985, -284.1341335259228913, -197.3122452978345507 ) ) ;
#85097=CARTESIAN_POINT ( 'NONE',  ( -73.83216537073211327, -284.1322001869087899, -206.4417270484278504 ) ) ;
#85098=CARTESIAN_POINT ( 'NONE',  ( 12.82642582302400491, -286.5808177466368534, -324.8470345085156055 ) ) ;
#85099=CARTESIAN_POINT ( 'NONE',  ( 33.34597996191038760, -283.0169606376890670, -290.1192147791099956 ) ) ;
#85100=CARTESIAN_POINT ( 'NONE',  ( -20.59804235624495306, -274.8371346787785114, -343.5215281646900962 ) ) ;
#85101=CARTESIAN_POINT ( 'NONE',  ( 28.02290218778222552, -285.4347668228930388, -231.0941579304074480 ) ) ;
#85102=CARTESIAN_POINT ( 'NONE',  ( -107.0396811834525721, -298.9146376407643970, -242.5232011649561343 ) ) ;
#85103=CARTESIAN_POINT ( 'NONE',  ( -72.72688878428748183, -283.5848898605697173, -203.9866864869890151 ) ) ;
#85104=CARTESIAN_POINT ( 'NONE',  ( -54.55969900859885513, -280.7668289612183230, -199.1262457046966290 ) ) ;
#85105=CARTESIAN_POINT ( 'NONE',  ( 24.82639920173008363, -288.9813564662231329, -228.0870313837762353 ) ) ;
#85108=CARTESIAN_POINT ( 'NONE',  ( 1.059069738076139355, -296.4639095254632934, -335.4356527227207039 ) ) ;
#85109=CARTESIAN_POINT ( 'NONE',  ( -90.88400694663341994, -277.2926712029276928, -217.7687666443969761 ) ) ;
#85110=CARTESIAN_POINT ( 'NONE',  ( -114.0260403342920767, -289.8102959298465748, -265.4958546589053867 ) ) ;
#85111=CARTESIAN_POINT ( 'NONE',  ( -63.87544708689493689, -293.8037395226788249, -339.2803606632087394 ) ) ;
#85112=CARTESIAN_POINT ( 'NONE',  ( -72.34997182512830705, -278.2633960628332375, -205.7417370536588521 ) ) ;
#85113=CARTESIAN_POINT ( 'NONE',  ( -79.65387282725808404, -271.5556788880574004, -209.0531563296729303 ) ) ;
#85114=CARTESIAN_POINT ( 'NONE',  ( 14.67709267725359723, -295.6162941855350823, -322.3488598585770433 ) ) ;
#85115=CARTESIAN_POINT ( 'NONE',  ( -69.91165696735023971, -288.1233781216987495, -202.8022627189028810 ) ) ;
#85116=CARTESIAN_POINT ( 'NONE',  ( -111.6352531339310730, -294.8115846643840428, -287.8296368892456485 ) ) ;
#85117=CARTESIAN_POINT ( 'NONE',  ( -15.59669151028512601, -290.3663005782199775, -340.9382469843984609 ) ) ;
#85118=CARTESIAN_POINT ( 'NONE',  ( -14.15406459776590964, -290.5885695910864115, -197.9435387665427584 ) ) ;
#85119=CARTESIAN_POINT ( 'NONE',  ( -108.9193483062363015, -291.7537852849898741, -287.4495702318347412 ) ) ;
#85121=CARTESIAN_POINT ( 'NONE',  ( -52.41299710682623214, -292.6571432814385503, -198.7167985291134471 ) ) ;
#85124=CARTESIAN_POINT ( 'NONE',  ( -109.1072627452599590, -292.0995016353652431, -243.4197103671865250 ) ) ;
#85125=CARTESIAN_POINT ( 'NONE',  ( 26.88952970955130795, -280.0995232924028073, -309.8649764031260929 ) ) ;
#85126=CARTESIAN_POINT ( 'NONE',  ( 19.34579087098954631, -292.9012003052814634, -224.3464744986668506 ) ) ;
#85127=CARTESIAN_POINT ( 'NONE',  ( 26.28061663383780555, -280.9790484413255172, -226.8952720309916913 ) ) ;
#85128=CARTESIAN_POINT ( 'NONE',  ( -102.9022936410183036, -283.6914472266286111, -310.7040587492527948 ) ) ;
#85129=CARTESIAN_POINT ( 'NONE',  ( -89.96800694927424047, -287.7974552624789908, -323.5635639376462791 ) ) ;
#85130=CARTESIAN_POINT ( 'NONE',  ( 26.20571468236173729, -279.1711639553267901, -231.8870890982719857 ) ) ;
#85131=CARTESIAN_POINT ( 'NONE',  ( -86.42140543987619594, -283.3709929050452843, -213.5809814034779777 ) ) ;
#85132=CARTESIAN_POINT ( 'NONE',  ( 1.042114091244876084, -279.0342162657594827, -204.3510423811589760 ) ) ;
#85133=CARTESIAN_POINT ( 'NONE',  ( 31.15191992416325917, -286.0267907822830011, -235.8630525147888477 ) ) ;
#85135=CARTESIAN_POINT ( 'NONE',  ( 34.22681023159566394, -295.3874046876959483, -288.3719131358678283 ) ) ;
#85136=CARTESIAN_POINT ( 'NONE',  ( 33.16280089125246633, -276.5983525594442085, -240.7674246092316821 ) ) ;
#85137=CARTESIAN_POINT ( 'NONE',  ( -104.2924725162575186, -277.8255362276186133, -299.6371340139624522 ) ) ;
#85138=CARTESIAN_POINT ( 'NONE',  ( -72.17416494254028692, -291.7709689234059169, -201.6755684035830143 ) ) ;
#85140=CARTESIAN_POINT ( 'NONE',  ( -67.33270816540002102, -281.5222478761535854, -339.7142263270876583 ) ) ;
#85141=EDGE_CURVE ( 'NONE', #41846, #16234, #77763, .T. ) ;
#85142=CARTESIAN_POINT ( 'NONE',  ( -110.2057910997127692, -289.7077302493710249, -262.9968329055291179 ) ) ;
#85144=CARTESIAN_POINT ( 'NONE',  ( -79.47973234395216480, -295.4833137047606328, -208.2552614602541610 ) ) ;
#85148=CARTESIAN_POINT ( 'NONE',  ( -37.54383090720561000, -291.5572420757261511, -197.2874045456559600 ) ) ;
#85150=CARTESIAN_POINT ( 'NONE',  ( -21.33282851196157992, -277.7666405000204577, -200.3683826091710216 ) ) ;
#85151=CARTESIAN_POINT ( 'NONE',  ( -79.35822855277511678, -294.6633583261095168, -334.6062076911250074 ) ) ;
#85152=CARTESIAN_POINT ( 'NONE',  ( 33.42520733454561110, -280.0399455443528041, -297.4230892120960448 ) ) ;
#85153=CARTESIAN_POINT ( 'NONE',  ( -108.8360934830187432, -285.5186513751361304, -297.7455786420215418 ) ) ;
#85154=CARTESIAN_POINT ( 'NONE',  ( 33.71080274108204833, -287.1638068335643084, -253.5577049223417418 ) ) ;
#85156=CARTESIAN_POINT ( 'NONE',  ( 28.66001379598199605, -277.5139176392491436, -303.2555014726411287 ) ) ;
#85157=CARTESIAN_POINT ( 'NONE',  ( -110.7644855535513244, -294.3978074591867085, -283.8834992514319424 ) ) ;
#85158=CARTESIAN_POINT ( 'NONE',  ( -110.0452475343240337, -298.4935408777866428, -256.4310379988921795 ) ) ;
#85159=CARTESIAN_POINT ( 'NONE',  ( -105.8795943025450441, -277.6976001720707359, -243.9569400051724983 ) ) ;
#85162=CARTESIAN_POINT ( 'NONE',  ( -113.1837907185554002, -296.0502194031610657, -283.8427757149162289 ) ) ;
#85163=CARTESIAN_POINT ( 'NONE',  ( 35.70180492342255718, -289.6588162466495646, -284.7784461973581642 ) ) ;
#85167=CARTESIAN_POINT ( 'NONE',  ( 34.86120687879893865, -288.3551833419904256, -281.8704210473467811 ) ) ;
#85169=CARTESIAN_POINT ( 'NONE',  ( -73.64376054616512590, -278.6411536812860845, -202.7076109665544834 ) ) ;
#85170=CARTESIAN_POINT ( 'NONE',  ( -113.0402375488554725, -297.3729904463028220, -256.8317344364228916 ) ) ;
#85171=CARTESIAN_POINT ( 'NONE',  ( -111.9216962285983499, -288.5211690208938649, -283.7810469209765643 ) ) ;
#85172=CARTESIAN_POINT ( 'NONE',  ( -99.98882173819012564, -296.2916962489630919, -315.1843537141244838 ) ) ;
#85173=CARTESIAN_POINT ( 'NONE',  ( 20.19693193804779341, -293.2516516346162234, -225.3809688278342662 ) ) ;
#85178=CARTESIAN_POINT ( 'NONE',  ( -74.07639917867282975, -291.0511989299233733, -337.2585403909363322 ) ) ;
#85179=CARTESIAN_POINT ( 'NONE',  ( 36.57525178469696669, -283.6233781216987495, -234.7283546768995564 ) ) ;
#85181=CARTESIAN_POINT ( 'NONE',  ( 33.46881879726637266, -281.2844262409695375, -300.4834513702567733 ) ) ;
#85182=CARTESIAN_POINT ( 'NONE',  ( -72.24187692466479405, -285.5151786685437401, -336.5578406255497725 ) ) ;
#85183=CARTESIAN_POINT ( 'NONE',  ( 36.12973860835963080, -285.8596019781211339, -249.1837030589231006 ) ) ;
#85184=CARTESIAN_POINT ( 'NONE',  ( -94.53073418536543215, -289.2952341018810216, -222.6890646630564561 ) ) ;
#85185=CARTESIAN_POINT ( 'NONE',  ( 36.42673736179660438, -277.1923038942890685, -253.0269380266633164 ) ) ;
#85188=CARTESIAN_POINT ( 'NONE',  ( -69.25141642484055637, -277.4839857884362573, -336.0314094350834466 ) ) ;
#85189=CARTESIAN_POINT ( 'NONE',  ( -5.506616776514092315, -279.8309826340072846, -204.5551901600002225 ) ) ;
#85190=CARTESIAN_POINT ( 'NONE',  ( -51.24304084389724778, -278.3055513681374009, -345.7815743271923452 ) ) ;
#85191=CARTESIAN_POINT ( 'NONE',  ( -111.4472420527611121, -277.1023955594365589, -289.8131474838088479 ) ) ;
#85192=CARTESIAN_POINT ( 'NONE',  ( 187.4789372167241766, 270.1634884999963901, -138.2063514411550500 ) ) ;
#85193=CARTESIAN_POINT ( 'NONE',  ( -107.8660944823039074, -273.8822899904735664, -239.9094819157917300 ) ) ;
#85194=CARTESIAN_POINT ( 'NONE',  ( -70.48996840331989233, -299.0489159655415961, -201.5149226909154550 ) ) ;
#85195=CARTESIAN_POINT ( 'NONE',  ( -95.99890600148557951, -293.6948066931273615, -223.6242672951989618 ) ) ;
#85196=CARTESIAN_POINT ( 'NONE',  ( 35.76128761417646729, -288.7123855299365687, -276.4935646971462688 ) ) ;
#85197=CARTESIAN_POINT ( 'NONE',  ( -95.06171104682378825, -286.9886611357956099, -220.8617912217218588 ) ) ;
#85198=CARTESIAN_POINT ( 'NONE',  ( 33.81144287587709840, -286.6791522105248760, -253.5402735174342581 ) ) ;
#85199=CARTESIAN_POINT ( 'NONE',  ( -67.86271102804410305, -282.9498239865104097, -340.9868554797391198 ) ) ;
#85200=CARTESIAN_POINT ( 'NONE',  ( 33.50826380960220519, -279.6817165435378456, -249.7038426051238389 ) ) ;
#85201=CARTESIAN_POINT ( 'NONE',  ( 25.99240659234478557, -288.8878690167856007, -231.6357205683218865 ) ) ;
#85202=CARTESIAN_POINT ( 'NONE',  ( 29.61062113970190168, -279.6190982408054992, -239.4476131005396837 ) ) ;
#85203=CARTESIAN_POINT ( 'NONE',  ( -99.58389348133435703, -279.3301550459626128, -309.5349483311418339 ) ) ;
#85204=CARTESIAN_POINT ( 'NONE',  ( 13.77886254513190778, -276.8043918556671770, -322.6300176060282183 ) ) ;
#85205=CARTESIAN_POINT ( 'NONE',  ( -73.00270171123558782, -288.3089333092536890, -338.1718296038213225 ) ) ;
#85206=CARTESIAN_POINT ( 'NONE',  ( -74.18954128489318123, -284.3315523653108130, -337.8474452113295570 ) ) ;
#85207=CARTESIAN_POINT ( 'NONE',  ( -113.4275307794020762, -285.1918653366378180, -258.5871256592184864 ) ) ;
#85208=CARTESIAN_POINT ( 'NONE',  ( 30.02067659130888444, -281.3414847057487691, -242.2308814531408245 ) ) ;
#85212=CARTESIAN_POINT ( 'NONE',  ( -93.80682671813032414, -293.1089328461043237, -219.8438440976675281 ) ) ;
#85213=CARTESIAN_POINT ( 'NONE',  ( -68.11494070989996885, -290.3412934247321573, -200.3018168022576333 ) ) ;
#85214=CARTESIAN_POINT ( 'NONE',  ( -108.1645366271926605, -271.8585874837364713, -251.5245032702783021 ) ) ;
#85215=CARTESIAN_POINT ( 'NONE',  ( 39.55438786971591014, -292.8642687002558773, -267.4487499859367290 ) ) ;
#85216=CARTESIAN_POINT ( 'NONE',  ( -92.94751270179145308, -288.3483522770085870, -318.7975232286609071 ) ) ;
#85217=CARTESIAN_POINT ( 'NONE',  ( 36.72188640440895568, -291.7975550469133168, -270.7878293311848665 ) ) ;
#85219=CARTESIAN_POINT ( 'NONE',  ( -26.40062462343085770, -290.1150390258587777, -342.9894628698535826 ) ) ;
#85222=CARTESIAN_POINT ( 'NONE',  ( -109.7098821290231285, -292.8061080222270220, -250.6184949141938034 ) ) ;
#85223=CARTESIAN_POINT ( 'NONE',  ( -111.8453999614888801, -288.6844786862233718, -260.0197317116807767 ) ) ;
#85224=CARTESIAN_POINT ( 'NONE',  ( -104.3897491143448377, -292.9974844449021703, -236.6378879720811881 ) ) ;
#85225=CARTESIAN_POINT ( 'NONE',  ( -39.99440614488874957, -286.9592598977974376, -197.1738813941064734 ) ) ;
#85226=CARTESIAN_POINT ( 'NONE',  ( 30.51958622879578087, -295.1264562719712785, -237.9157287464351782 ) ) ;
#85230=CARTESIAN_POINT ( 'NONE',  ( 37.67724985461494924, -277.4344160468858718, -262.7214806844898476 ) ) ;
#85231=CARTESIAN_POINT ( 'NONE',  ( -101.4990905596771853, -295.1910754121335003, -312.7419710783055393 ) ) ;
#85232=CARTESIAN_POINT ( 'NONE',  ( 36.38978654180912997, -273.7007394384947361, -263.3466997308307782 ) ) ;
#85233=CARTESIAN_POINT ( 'NONE',  ( -98.07443147968626818, -276.0423527495618146, -313.4280044050193510 ) ) ;
#85234=CARTESIAN_POINT ( 'NONE',  ( -109.9779857038130473, -273.9000898063000022, -259.4728672392996032 ) ) ;
#85235=CARTESIAN_POINT ( 'NONE',  ( 26.44872250418129411, -273.5695005989383048, -228.2970207857106573 ) ) ;
#85238=CARTESIAN_POINT ( 'NONE',  ( -110.6389399451682607, -298.0703472837783465, -263.2607094851260854 ) ) ;
#85240=CARTESIAN_POINT ( 'NONE',  ( -103.8696764246535480, -297.7660619708098579, -239.7985426181126911 ) ) ;
#85242=CARTESIAN_POINT ( 'NONE',  ( 33.32080440664549315, -285.2341006420001577, -244.1844632316892785 ) ) ;
#85243=CARTESIAN_POINT ( 'NONE',  ( -94.61138920322240153, -273.0242730988997550, -225.0932185639196064 ) ) ;
#85245=CARTESIAN_POINT ( 'NONE',  ( -2.222905909516156964, -286.5039514251818105, -201.8214042656358913 ) ) ;
#85246=CARTESIAN_POINT ( 'NONE',  ( -95.44513266483720315, -289.5361669816564358, -320.8560228644030872 ) ) ;
#85247=CARTESIAN_POINT ( 'NONE',  ( -99.41050082484480299, -299.1087069299199470, -227.6082222131907145 ) ) ;
#85248=CARTESIAN_POINT ( 'NONE',  ( 34.87951317196877454, -291.8051198922510139, -290.0088780720487875 ) ) ;
#85249=CARTESIAN_POINT ( 'NONE',  ( 39.47964225627480772, -280.7081309644808016, -267.0745029167381404 ) ) ;
#85250=CARTESIAN_POINT ( 'NONE',  ( -114.2704648735229114, -294.0523547857347353, -270.3284710469133074 ) ) ;
#85252=CARTESIAN_POINT ( 'NONE',  ( -3.195244146020708609, -287.3858593435825242, -335.3877774959526050 ) ) ;
#85254=CARTESIAN_POINT ( 'NONE',  ( -2.458236550231002404, -286.5909035662497217, -336.8124834570580219 ) ) ;
#85255=CARTESIAN_POINT ( 'NONE',  ( -110.5769288073768308, -274.1794891676080965, -262.1569097855852419 ) ) ;
#85256=CARTESIAN_POINT ( 'NONE',  ( 12.59329519745948822, -282.1578373837249387, -212.5242566118509160 ) ) ;
#85257=CARTESIAN_POINT ( 'NONE',  ( -112.5929422392180044, -294.5103187762870220, -275.2079067232778016 ) ) ;
#85258=CARTESIAN_POINT ( 'NONE',  ( 20.18097106163576626, -282.1856796499242819, -315.3071111209888500 ) ) ;
#85259=CARTESIAN_POINT ( 'NONE',  ( -114.3379842354461147, -296.7282924929146475, -269.6046537453748329 ) ) ;
#85260=CARTESIAN_POINT ( 'NONE',  ( -96.76785638608127726, -274.5813251528768433, -226.8724341962961262 ) ) ;
#85261=CARTESIAN_POINT ( 'NONE',  ( -7.061807674329386941, -282.4495544396286277, -201.7314135402912143 ) ) ;
#85262=CARTESIAN_POINT ( 'NONE',  ( -68.13556585643250685, -296.6963354173360017, -203.9008431247150099 ) ) ;
#85265=CARTESIAN_POINT ( 'NONE',  ( -48.55135453237547694, -285.1754691331672689, -344.1594272355102362 ) ) ;
#85267=CARTESIAN_POINT ( 'NONE',  ( 10.59707575819633618, -291.9094976428776818, -330.5268031993606428 ) ) ;
#85268=CARTESIAN_POINT ( 'NONE',  ( 38.02199148988064081, -274.9370930083411508, -285.3435345675689518 ) ) ;
#85269=CARTESIAN_POINT ( 'NONE',  ( 4.505380487589857985, -292.4674454044224490, -210.4842547104564687 ) ) ;
#85270=CARTESIAN_POINT ( 'NONE',  ( 18.13949038304979666, -283.7577681207872047, -318.8641617330839608 ) ) ;
#85271=CARTESIAN_POINT ( 'NONE',  ( 33.28788691199553540, -277.4330673097487079, -291.8036074388513157 ) ) ;
#85272=CARTESIAN_POINT ( 'NONE',  ( -63.69166261321188216, -284.8143236728391230, -342.0847944742351956 ) ) ;
#85273=CARTESIAN_POINT ( 'NONE',  ( -106.5532703262639700, -283.0219064618000857, -294.9438690124823097 ) ) ;
#85274=CARTESIAN_POINT ( 'NONE',  ( -26.20972853582104989, -298.1879210266415612, -193.3611172013085024 ) ) ;
#85275=CARTESIAN_POINT ( 'NONE',  ( 5.869528243787705435, -276.3170591412307999, -334.0932899766542050 ) ) ;
#85276=CARTESIAN_POINT ( 'NONE',  ( -7.386843470316971860, -296.5764373502184981, -338.5220181679449638 ) ) ;
#85280=CARTESIAN_POINT ( 'NONE',  ( -106.6336108941719942, -295.0905608128484801, -239.5894245375911282 ) ) ;
#85281=CARTESIAN_POINT ( 'NONE',  ( 20.06692595758643094, -275.6969610454101485, -315.5723923917195748 ) ) ;
#85283=CARTESIAN_POINT ( 'NONE',  ( 38.16294094168111428, -294.9285504027546381, -258.9728401621232479 ) ) ;
#85284=CARTESIAN_POINT ( 'NONE',  ( 35.07219688184650863, -294.4388301522570828, -245.2159277609581522 ) ) ;
#85285=CARTESIAN_POINT ( 'NONE',  ( -110.1278127687702977, -292.3285804350342119, -287.7453130306989237 ) ) ;
#85286=CARTESIAN_POINT ( 'NONE',  ( -103.4890587661245860, -276.0870243290940493, -305.3547655319710543 ) ) ;
#85288=CARTESIAN_POINT ( 'NONE',  ( -110.0178722561057612, -280.6813831034252757, -254.1940392802580106 ) ) ;
#85289=CARTESIAN_POINT ( 'NONE',  ( -78.77108140683492365, -293.6945354681253093, -332.2693337293206355 ) ) ;
#85290=CARTESIAN_POINT ( 'NONE',  ( 37.03749106470723973, -283.2292351932150609, -255.9374776507845581 ) ) ;
#85291=CARTESIAN_POINT ( 'NONE',  ( -71.30928882695380366, -284.5128416489520760, -205.3962890952580551 ) ) ;
#85292=CARTESIAN_POINT ( 'NONE',  ( -87.93210667360744992, -231.3106068285471224, -347.0561263492803619 ) ) ;
#85294=CARTESIAN_POINT ( 'NONE',  ( -109.5199196913323050, -284.0686913048139104, -281.7487380331803024 ) ) ;
#85296=CARTESIAN_POINT ( 'NONE',  ( 39.33101504801366843, -282.5903319552435278, -267.0569256189247653 ) ) ;
#85298=CARTESIAN_POINT ( 'NONE',  ( -73.41240170980816515, -284.3798461233395756, -202.7234327738455306 ) ) ;
#85300=CARTESIAN_POINT ( 'NONE',  ( -112.5606587759765205, -279.3003077765673083, -285.7534072906063329 ) ) ;
#85301=CARTESIAN_POINT ( 'NONE',  ( -113.5386302917111152, -280.0206454456625238, -274.4520328841388732 ) ) ;
#85302=CARTESIAN_POINT ( 'NONE',  ( -84.51095865778017924, -280.0735979586750659, -209.5617438996513897 ) ) ;
#85303=CARTESIAN_POINT ( 'NONE',  ( -92.05005921254146983, -270.6952119285918457, -226.6919474004047572 ) ) ;
#85304=CARTESIAN_POINT ( 'NONE',  ( 186.5495922466713239, 262.9189426707559960, -153.3149145016442105 ) ) ;
#85306=CARTESIAN_POINT ( 'NONE',  ( -21.57191473664897075, -276.2549749433813986, -197.2082486465691602 ) ) ;
#85307=CARTESIAN_POINT ( 'NONE',  ( -100.3960620948416960, -247.6577473148603303, -334.0155409199911105 ) ) ;
#85309=CARTESIAN_POINT ( 'NONE',  ( -60.21417990973924361, -277.7744246008469418, -199.2524386249262989 ) ) ;
#85310=CARTESIAN_POINT ( 'NONE',  ( 37.61051428378693373, -295.4716490251918231, -282.9356773867759784 ) ) ;
#85311=CARTESIAN_POINT ( 'NONE',  ( 35.74349899309140710, -292.9421053615432697, -273.5016115750136692 ) ) ;
#85312=CARTESIAN_POINT ( 'NONE',  ( -97.24611791307208364, -289.4118717051399017, -318.6621994282728565 ) ) ;
#85314=CARTESIAN_POINT ( 'NONE',  ( 19.08222239640173257, -292.8335499964741189, -321.9643450534176168 ) ) ;
#85315=CARTESIAN_POINT ( 'NONE',  ( -95.57589920714340792, -283.5841081472163410, -225.0060873182454202 ) ) ;
#85316=CARTESIAN_POINT ( 'NONE',  ( -60.66921659047097393, -293.6068536820058625, -199.8324090037635585 ) ) ;
#85317=CARTESIAN_POINT ( 'NONE',  ( -97.92946719213840368, -285.2910866066442850, -312.0474536373212686 ) ) ;
#85319=CARTESIAN_POINT ( 'NONE',  ( -42.05153703266179122, -292.9353947670043112, -193.7410315202664606 ) ) ;
#85320=CARTESIAN_POINT ( 'NONE',  ( 21.86548535142082983, -282.6430840897753001, -313.1902230019342142 ) ) ;
#85321=CARTESIAN_POINT ( 'NONE',  ( 17.26765468212770926, -293.0891392166258811, -324.1564427928163354 ) ) ;
#85323=CARTESIAN_POINT ( 'NONE',  ( -38.90661529880382830, -289.8741459623522019, -347.1837049061523430 ) ) ;
#85324=CARTESIAN_POINT ( 'NONE',  ( -69.32599892440725853, -289.9541410488120050, -340.3507502568501195 ) ) ;
#85325=CARTESIAN_POINT ( 'NONE',  ( 33.02870052079136798, -287.4622644176563995, -250.9444571718619272 ) ) ;
#85328=CARTESIAN_POINT ( 'NONE',  ( -97.83368150893323900, -295.8665948216546440, -223.4996305552631384 ) ) ;
#85329=CARTESIAN_POINT ( 'NONE',  ( 33.34382439534415710, -280.3580891893270177, -251.1567770347494672 ) ) ;
#85330=CARTESIAN_POINT ( 'NONE',  ( -64.87220129343742769, -273.2097151345325869, -198.5026791848366656 ) ) ;
#85331=CARTESIAN_POINT ( 'NONE',  ( -18.05753358120802687, -293.2788770718879050, -341.4865611886954753 ) ) ;
#85332=CARTESIAN_POINT ( 'NONE',  ( 36.02203325793278310, -277.1849917597225499, -260.5766079305047924 ) ) ;
#85333=CARTESIAN_POINT ( 'NONE',  ( -39.17121545107871583, -296.2687728475834206, -196.3578148628117788 ) ) ;
#85334=CARTESIAN_POINT ( 'NONE',  ( -9.063793263993545679, -295.8790172259487576, -338.1058149697218482 ) ) ;
#85335=CARTESIAN_POINT ( 'NONE',  ( -63.66720964127983962, -296.4831069969220039, -338.8341469933401982 ) ) ;
#85337=CARTESIAN_POINT ( 'NONE',  ( -90.14289132493765067, -297.3833651113022256, -325.3743899141696829 ) ) ;
#85338=CARTESIAN_POINT ( 'NONE',  ( -107.1756566770312702, -294.9149607304752863, -242.4140483279979037 ) ) ;
#85339=CARTESIAN_POINT ( 'NONE',  ( -17.41276450388166808, -292.9674788075290621, -199.9754590976942552 ) ) ;
#85340=CARTESIAN_POINT ( 'NONE',  ( -14.85548855148504188, -298.9781657277604268, -193.4606360843729647 ) ) ;
#85341=CARTESIAN_POINT ( 'NONE',  ( -107.5194736246562570, -288.8336646049432943, -292.6760122069681529 ) ) ;
#85342=CARTESIAN_POINT ( 'NONE',  ( -43.67574994848473580, -275.9724079498772653, -195.5769595042413584 ) ) ;
#85343=CARTESIAN_POINT ( 'NONE',  ( -114.2803945993239978, -273.0802817338963564, -267.5021993077760953 ) ) ;
#85345=CARTESIAN_POINT ( 'NONE',  ( -94.78744396980151521, -296.2499511348794954, -315.4396494731284974 ) ) ;
#85347=CARTESIAN_POINT ( 'NONE',  ( -64.18059975866478339, -281.6837639149981101, -199.8924440197786225 ) ) ;
#85348=CARTESIAN_POINT ( 'NONE',  ( 25.88259953915978784, -279.6640866499496383, -227.1874935540791682 ) ) ;
#85349=CARTESIAN_POINT ( 'NONE',  ( 15.67724591466546791, -281.6736722920717853, -326.0594496172246863 ) ) ;
#85350=CARTESIAN_POINT ( 'NONE',  ( 10.45620175047695177, -275.7607702168896822, -330.6675780036783294 ) ) ;
#85351=CARTESIAN_POINT ( 'NONE',  ( 20.47257553036742195, -279.2748433380169786, -220.7030801668565516 ) ) ;
#85352=CARTESIAN_POINT ( 'NONE',  ( 36.34319700263598207, -279.7422620152529475, -285.2125275018509569 ) ) ;
#85353=CARTESIAN_POINT ( 'NONE',  ( 7.705813286384870509, -273.2558397446632057, -212.1709431193758917 ) ) ;
#85354=CARTESIAN_POINT ( 'NONE',  ( -46.01798673481732749, -279.1622160332308908, -344.9091645557127208 ) ) ;
#85357=CARTESIAN_POINT ( 'NONE',  ( -97.41883034708538958, -295.4216997323484293, -223.8136569756578638 ) ) ;
#85358=CARTESIAN_POINT ( 'NONE',  ( -11.68895326348806485, -290.4045086914899798, -199.4518877087343185 ) ) ;
#85359=CARTESIAN_POINT ( 'NONE',  ( -33.53936521356042277, -292.0987747743462819, -193.4550567832122852 ) ) ;
#85360=CARTESIAN_POINT ( 'NONE',  ( 37.72185028693903774, -277.4904424940166336, -265.5315688099045701 ) ) ;
#85361=CARTESIAN_POINT ( 'NONE',  ( 1.674055110504922395, -272.5737339518336171, -206.3082375524538179 ) ) ;
#85363=CARTESIAN_POINT ( 'NONE',  ( 35.10516137891819710, -283.7488129434112807, -292.0067881129322700 ) ) ;
#85365=CARTESIAN_POINT ( 'NONE',  ( -111.0247452101357908, -282.7325274017208585, -256.3006823243030112 ) ) ;
#85367=CARTESIAN_POINT ( 'NONE',  ( -6.612568104887075471, -293.4343224025716950, -337.0158323780170804 ) ) ;
#85368=CARTESIAN_POINT ( 'NONE',  ( 33.01875402797421089, -285.3825332752226132, -246.6910531174620473 ) ) ;
#85370=CARTESIAN_POINT ( 'NONE',  ( -7.207478984242021269, -292.6567565507618838, -339.0549699003111073 ) ) ;
#85371=CARTESIAN_POINT ( 'NONE',  ( -61.03494739089646970, -281.8339807779076409, -342.9513861241897530 ) ) ;
#85372=CARTESIAN_POINT ( 'NONE',  ( -39.74750515157573005, -281.6216008673962961, -196.5876821948639304 ) ) ;
#85373=CARTESIAN_POINT ( 'NONE',  ( -106.3282113879519244, -286.1866761557398036, -237.0614185597411563 ) ) ;
#85374=CARTESIAN_POINT ( 'NONE',  ( 31.11837850745464351, -279.3620110375047147, -237.2674021643780122 ) ) ;
#85375=CARTESIAN_POINT ( 'NONE',  ( -4.594561174994372443, -286.4961386153739227, -205.1183031261544443 ) ) ;
#85376=AXIS2_PLACEMENT_3D ( 'NONE', #40785, #31854, #46049 ) ;
#85377=CARTESIAN_POINT ( 'NONE',  ( -110.9410942854753586, -280.0095523428630599, -267.9065712911786932 ) ) ;
#85378=CARTESIAN_POINT ( 'NONE',  ( -106.6008990167036359, -279.6694388792457744, -246.6308072624681245 ) ) ;
#85379=CARTESIAN_POINT ( 'NONE',  ( -84.50354520639299949, -287.3862664607104307, -211.5889547711989280 ) ) ;
#85380=ORIENTED_EDGE ( 'NONE', *, *, #46511, .F. ) ;
#85381=CARTESIAN_POINT ( 'NONE',  ( -97.34501241894210466, -297.0321885429960957, -222.1055222587203275 ) ) ;
#85382=CARTESIAN_POINT ( 'NONE',  ( -53.74600324994583644, -291.2436144459783236, -343.1810715573777202 ) ) ;
#85384=CARTESIAN_POINT ( 'NONE',  ( 36.60358173371528068, -290.4805209788416391, -305.9350535429201159 ) ) ;
#85386=CARTESIAN_POINT ( 'NONE',  ( -29.99218240839089233, -272.1448144039434851, -195.5546141523136043 ) ) ;
#85387=CARTESIAN_POINT ( 'NONE',  ( 38.91108047583755081, -291.9516414418151271, -270.3308287414987490 ) ) ;
#85388=CARTESIAN_POINT ( 'NONE',  ( -69.27878068144187296, -297.1278496948397105, -204.6495411668220754 ) ) ;
#85389=CARTESIAN_POINT ( 'NONE',  ( -10.45325000053184006, -290.2151086143339853, -339.0286747491756500 ) ) ;
#85391=CARTESIAN_POINT ( 'NONE',  ( -30.18642673180180580, -281.9039182815166669, -196.6434089596836827 ) ) ;
#85392=CARTESIAN_POINT ( 'NONE',  ( -72.88356861356207617, -290.9388561554251851, -338.0173291965904241 ) ) ;
#85393=CARTESIAN_POINT ( 'NONE',  ( -112.3810011312560704, -291.6787743110392626, -285.3405846625454956 ) ) ;
#85394=CARTESIAN_POINT ( 'NONE',  ( -75.76605108457408733, -287.5393609507518136, -205.9517250169661224 ) ) ;
#85395=CARTESIAN_POINT ( 'NONE',  ( -71.23650637898326465, -279.7836696436721127, -201.2225461593754687 ) ) ;
#85396=CARTESIAN_POINT ( 'NONE',  ( -19.64864832398396643, -292.9063518290886350, -343.8742824224568153 ) ) ;
#85397=CARTESIAN_POINT ( 'NONE',  ( 38.79505494141974964, -281.2373538934267572, -258.5176527606635091 ) ) ;
#85398=CARTESIAN_POINT ( 'NONE',  ( 36.33497591933855375, -277.5358108856356125, -279.8612989999423917 ) ) ;
#85399=CARTESIAN_POINT ( 'NONE',  ( 34.45848030099739390, -278.0519495502701375, -270.3284710469131937 ) ) ;
#85400=CARTESIAN_POINT ( 'NONE',  ( 37.18408174626422635, -273.9799391725375699, -285.1895316596790053 ) ) ;
#85402=CARTESIAN_POINT ( 'NONE',  ( 30.08069009637267399, -280.6825635611310190, -242.2148973141834460 ) ) ;
#85403=CARTESIAN_POINT ( 'NONE',  ( -110.2838281678035912, -279.4595696811803691, -293.9295440567838114 ) ) ;
#85404=CARTESIAN_POINT ( 'NONE',  ( -24.52679693562780017, -275.5341701822347886, -197.9419132277197662 ) ) ;
#85405=CARTESIAN_POINT ( 'NONE',  ( -114.0908887220844150, -283.6516562711590836, -267.1123721748851949 ) ) ;
#85406=CARTESIAN_POINT ( 'NONE',  ( -106.6675788237325548, -292.6550733738876033, -244.2946033630293527 ) ) ;
#85407=CARTESIAN_POINT ( 'NONE',  ( -32.75137001562904970, -275.7091857408825604, -194.2864888338620517 ) ) ;
#85408=CARTESIAN_POINT ( 'NONE',  ( -108.7126526473435035, -274.2203027110222138, -242.6564437103182854 ) ) ;
#85410=CARTESIAN_POINT ( 'NONE',  ( -110.2692839601484565, -298.7682539721303101, -253.5802971519963194 ) ) ;
#85411=CARTESIAN_POINT ( 'NONE',  ( -72.28702149830643009, -281.5155043557019212, -336.5340198642109613 ) ) ;
#85412=CARTESIAN_POINT ( 'NONE',  ( -86.49626782610978637, -291.0578643194762662, -211.0502616425293638 ) ) ;
#85413=CARTESIAN_POINT ( 'NONE',  ( 30.64214181755867017, -273.9785493321141985, -301.1839023142103429 ) ) ;
#85414=CARTESIAN_POINT ( 'NONE',  ( 5.128514372995561565, -290.0883040165365969, -333.6281812478321740 ) ) ;
#85415=CARTESIAN_POINT ( 'NONE',  ( -108.0275319073851392, -289.2145424529018101, -289.9838342090316701 ) ) ;
#85417=CARTESIAN_POINT ( 'NONE',  ( -110.6616201043788408, -289.3988017178612608, -248.8484327011938717 ) ) ;
#85418=CARTESIAN_POINT ( 'NONE',  ( -88.67894768929343741, -289.4640659242472793, -322.2896698550895280 ) ) ;
#85420=CARTESIAN_POINT ( 'NONE',  ( 1.353790694844288822, -287.6360598240672175, -204.1329171591973761 ) ) ;
#85421=CARTESIAN_POINT ( 'NONE',  ( -104.2890772281016325, -278.4919913213654468, -299.6448968440159888 ) ) ;
#85422=CARTESIAN_POINT ( 'NONE',  ( -27.79998188165951589, -293.8541569591969846, -346.5091900082400116 ) ) ;
#85423=CARTESIAN_POINT ( 'NONE',  ( -108.1300546628084192, -284.8191650665347083, -300.5359739669268038 ) ) ;
#85424=CARTESIAN_POINT ( 'NONE',  ( -95.80328488195675618, -285.5620326133076787, -220.2013545995151560 ) ) ;
#85425=CARTESIAN_POINT ( 'NONE',  ( 29.33549912996144116, -282.2876754222617706, -300.2550449009398221 ) ) ;
#85426=CARTESIAN_POINT ( 'NONE',  ( 103.2429438805325930, 116.4356071745880996, -282.9982326746781496 ) ) ;
#85427=CARTESIAN_POINT ( 'NONE',  ( -113.0914918815083325, -269.8132127191667564, -296.0580370876392067 ) ) ;
#85428=CARTESIAN_POINT ( 'NONE',  ( 137.7094901139326737, 178.8809403604650754, -238.3456290536556423 ) ) ;
#85429=CARTESIAN_POINT ( 'NONE',  ( 35.86023183603892761, -274.7655933550383907, -271.5978758200953962 ) ) ;
#85430=CARTESIAN_POINT ( 'NONE',  ( -5.160002530986704805, -273.4063308220990507, -204.4794539677491514 ) ) ;
#85431=CARTESIAN_POINT ( 'NONE',  ( -96.46815393572545361, -295.3969160455825431, -319.6115696248878066 ) ) ;
#85432=CARTESIAN_POINT ( 'NONE',  ( -29.67131002704720188, -125.4300734434975766, -360.8905850898509584 ) ) ;
#85433=CARTESIAN_POINT ( 'NONE',  ( -2.765335570163358181, -273.1843892286717619, -202.0986268218431405 ) ) ;
#85434=CARTESIAN_POINT ( 'NONE',  ( -78.21144900091205443, -299.3569442172352524, -208.3273320104813138 ) ) ;
#85435=CARTESIAN_POINT ( 'NONE',  ( -64.19759731154091753, -292.7730358496651775, -202.1347207499361218 ) ) ;
#85436=VERTEX_POINT ( 'NONE', #34162 ) ;
#85437=CARTESIAN_POINT ( 'NONE',  ( -80.50266295016409401, -298.4242525308100653, -206.8153012810754490 ) ) ;
#85438=CARTESIAN_POINT ( 'NONE',  ( 35.18605994602095421, -288.1606946722600355, -279.1765850866558480 ) ) ;
#85439=CARTESIAN_POINT ( 'NONE',  ( 37.60153573046810038, -294.1417491567841580, -253.3413171082922304 ) ) ;
#85440=CARTESIAN_POINT ( 'NONE',  ( -41.93561398675245755, -295.6007914749510519, -347.2146602143050700 ) ) ;
#85441=CARTESIAN_POINT ( 'NONE',  ( 34.83830210746106815, -293.8671038216530178, -281.6008562030149847 ) ) ;
#85444=CARTESIAN_POINT ( 'NONE',  ( 24.94344187158408488, -276.8966981663572824, -227.5611537256123995 ) ) ;
#85445=VERTEX_POINT ( 'NONE', #4333 ) ;
#85446=CARTESIAN_POINT ( 'NONE',  ( -77.45507643787013308, -279.0372459774230265, -204.6454729271333974 ) ) ;
#85448=CARTESIAN_POINT ( 'NONE',  ( -11.41811196136254303, -275.3394539857553696, -201.8132811880556403 ) ) ;
#85449=CARTESIAN_POINT ( 'NONE',  ( 38.54093798138981697, -277.2504618690291522, -265.4822052030980899 ) ) ;
#85450=CARTESIAN_POINT ( 'NONE',  ( -61.89442254362924700, -275.3896969983617851, -341.6592695692138477 ) ) ;
#85451=CARTESIAN_POINT ( 'NONE',  ( -98.53744200381302676, -297.7580489460414697, -230.2823291423905800 ) ) ;
#85452=CARTESIAN_POINT ( 'NONE',  ( -104.4815924179346212, -294.7228439471268757, -300.6123129739608544 ) ) ;
#85454=CARTESIAN_POINT ( 'NONE',  ( -100.2023290044299557, -279.6319692578316563, -225.9982028329368404 ) ) ;
#85455=EDGE_CURVE ( 'NONE', #82501, #38497, #39938, .T. ) ;
#85456=CARTESIAN_POINT ( 'NONE',  ( 22.46705677812836655, -276.3035800437105536, -312.3037599124360781 ) ) ;
#85457=CARTESIAN_POINT ( 'NONE',  ( 11.77389624498925258, -285.4022830271741213, -211.6323089209319619 ) ) ;
#85458=CARTESIAN_POINT ( 'NONE',  ( -35.55276828753007834, -300.0746522698417493, -195.1938344133556313 ) ) ;
#85460=CARTESIAN_POINT ( 'NONE',  ( 30.11461380323548198, -286.3685355557229855, -241.9059047431724423 ) ) ;
#85461=CARTESIAN_POINT ( 'NONE',  ( -46.56075853841169021, -278.1735434440051904, -196.8723759676163354 ) ) ;
#85462=CARTESIAN_POINT ( 'NONE',  ( -109.7082703757403976, -277.3016884326154923, -257.0024343338664607 ) ) ;
#85463=CARTESIAN_POINT ( 'NONE',  ( -74.53711531305629023, -281.6304886815091777, -334.9009908338637160 ) ) ;
#85464=CARTESIAN_POINT ( 'NONE',  ( 17.01494065473467998, -288.8269988651681501, -218.6671186982148640 ) ) ;
#85465=CARTESIAN_POINT ( 'NONE',  ( -40.50761639806828640, -278.2978907447136976, -343.7024132494160540 ) ) ;
#85467=CARTESIAN_POINT ( 'NONE',  ( -107.7263555860935611, -276.4235023735220125, -298.9963111501773483 ) ) ;
#85468=CARTESIAN_POINT ( 'NONE',  ( -0.5020590240191551423, -275.2071284404660787, -207.2059222955260509 ) ) ;
#85469=CARTESIAN_POINT ( 'NONE',  ( 24.75141919173618277, -282.9788861606731984, -227.9091212399665096 ) ) ;
#85471=CARTESIAN_POINT ( 'NONE',  ( -7.466347824704368641, -290.5836748055257317, -339.7781022376486249 ) ) ;
#85472=CARTESIAN_POINT ( 'NONE',  ( -107.1503436277639310, -294.9104573035562566, -242.8028733357952831 ) ) ;
#85473=CARTESIAN_POINT ( 'NONE',  ( 82.15976772225275226, -298.6975972703625644, -197.1770246269288691 ) ) ;
#85474=CARTESIAN_POINT ( 'NONE',  ( 20.25235203416342955, -273.5967206732531167, -224.6882792085102949 ) ) ;
#85475=CARTESIAN_POINT ( 'NONE',  ( 19.43636954527508465, -291.0236384560634519, -222.5373133760767814 ) ) ;
#85476=CARTESIAN_POINT ( 'NONE',  ( 88.37812178648184158, 82.46720509654242903, -304.8213980281626618 ) ) ;
#85478=CARTESIAN_POINT ( 'NONE',  ( -105.8991785296611141, -288.5965288166284495, -303.9862092998071148 ) ) ;
#85479=CARTESIAN_POINT ( 'NONE',  ( -103.7234390054959192, -285.7190485944348666, -302.7259751915948982 ) ) ;
#85480=CARTESIAN_POINT ( 'NONE',  ( 29.25440886013337050, -285.3105775831259052, -233.6604594917863551 ) ) ;
#85481=CARTESIAN_POINT ( 'NONE',  ( -110.0779476705021978, -285.8269609341642195, -281.8595101528047735 ) ) ;
#85482=CARTESIAN_POINT ( 'NONE',  ( -109.3537821472749556, -285.5259432252710212, -257.3730876721704135 ) ) ;
#85483=CARTESIAN_POINT ( 'NONE',  ( -53.07113772343158331, -293.8315063285199358, -196.6125193458454703 ) ) ;
#85484=CARTESIAN_POINT ( 'NONE',  ( 32.83754504310024203, -273.9956657480891522, -298.5054196352234044 ) ) ;
#85485=CARTESIAN_POINT ( 'NONE',  ( 39.35979346878447416, -275.9671065084103816, -276.8899135430260685 ) ) ;
#85486=CARTESIAN_POINT ( 'NONE',  ( -112.9276973838095159, -288.6573999724478767, -268.3678348825804960 ) ) ;
#85487=CARTESIAN_POINT ( 'NONE',  ( -84.86637858723672423, -277.6867629155370309, -331.0127353505313863 ) ) ;
#85488=CARTESIAN_POINT ( 'NONE',  ( -110.3939595230142743, -298.7306801683519097, -254.9628638157828107 ) ) ;
#85491=CARTESIAN_POINT ( 'NONE',  ( -88.02255192507298887, -284.0097323557801019, -217.1380521336927529 ) ) ;
#85492=CARTESIAN_POINT ( 'NONE',  ( -22.92500629182146454, -278.2362999985753049, -196.7069129976315196 ) ) ;
#85494=CARTESIAN_POINT ( 'NONE',  ( 23.93477325718336601, -273.4219383265481724, -224.8869322975220086 ) ) ;
#85495=CARTESIAN_POINT ( 'NONE',  ( -74.07165735627216918, -276.9027617096418226, -333.5655712296564843 ) ) ;
#85496=CARTESIAN_POINT ( 'NONE',  ( -50.57690759279955017, -296.7443813451467918, -342.8562008094031057 ) ) ;
#85497=CARTESIAN_POINT ( 'NONE',  ( 37.56064306032777722, -280.6800082276840271, -286.8877868902635555 ) ) ;
#85498=CARTESIAN_POINT ( 'NONE',  ( -31.57189788777413497, -295.9189228475019036, -343.4190485551495726 ) ) ;
#85499=CARTESIAN_POINT ( 'NONE',  ( -61.42036995063765659, -296.6735375929934548, -343.0354728500914234 ) ) ;
#85500=CARTESIAN_POINT ( 'NONE',  ( -109.6030553722883809, -272.3619811233771202, -259.5093225255930633 ) ) ;
#85501=CARTESIAN_POINT ( 'NONE',  ( -85.12225379204525666, -293.3926104201368048, -212.5509170035166164 ) ) ;
#85502=CARTESIAN_POINT ( 'NONE',  ( -113.8198857466201162, -284.8307530452827905, -261.4119767391071036 ) ) ;
#85503=CARTESIAN_POINT ( 'NONE',  ( -43.91165069348464556, -272.1096668562589116, -194.8292561368286044 ) ) ;
#85504=CARTESIAN_POINT ( 'NONE',  ( 37.37734162407514305, -287.1527367308601697, -251.7583008795115234 ) ) ;
#85505=CARTESIAN_POINT ( 'NONE',  ( -43.92062934987458078, -281.9486143028269112, -195.9554349219983749 ) ) ;
#85506=CARTESIAN_POINT ( 'NONE',  ( -19.74775943112968690, -285.3427172996281342, -199.2706003438800906 ) ) ;
#85507=CARTESIAN_POINT ( 'NONE',  ( -41.67124161301421026, -287.1065093832526713, -345.2489305224974601 ) ) ;
#85508=CARTESIAN_POINT ( 'NONE',  ( -106.3535322092011199, -272.9508360837029954, -295.9465859460973434 ) ) ;
#85509=CARTESIAN_POINT ( 'NONE',  ( 25.00649936477236679, -286.5354849934403205, -232.2731873275983219 ) ) ;
#85510=CARTESIAN_POINT ( 'NONE',  ( 28.11067463113290543, -283.0201968156267185, -310.5718127627725380 ) ) ;
#85511=CARTESIAN_POINT ( 'NONE',  ( -113.7713662134438977, -289.7076530896669624, -262.6486439669167794 ) ) ;
#85512=CARTESIAN_POINT ( 'NONE',  ( -99.60716562036697042, -280.7395715522028468, -226.4355875573334629 ) ) ;
#85513=CARTESIAN_POINT ( 'NONE',  ( -86.50075231068633741, -280.7013072837039545, -211.6687999738819315 ) ) ;
#85514=CARTESIAN_POINT ( 'NONE',  ( 31.07104722411070341, -281.0440341837937126, -244.7465731184199740 ) ) ;
#85515=CARTESIAN_POINT ( 'NONE',  ( 36.33353319184841723, -277.3721129037020319, -256.3268511106654159 ) ) ;
#85516=CARTESIAN_POINT ( 'NONE',  ( -4.502533278418947127, -294.6313252199440171, -340.0217587359314280 ) ) ;
#85517=CARTESIAN_POINT ( 'NONE',  ( -87.86071224173032590, -287.7820920545598824, -325.3828414447040132 ) ) ;
#85519=CARTESIAN_POINT ( 'NONE',  ( -96.34094964446404674, -296.0800069474249767, -226.8276945445428225 ) ) ;
#85520=VERTEX_POINT ( 'NONE', #62104 ) ;
#85521=CARTESIAN_POINT ( 'NONE',  ( 34.72362051837087904, -283.7143713935473102, -289.0641358370465923 ) ) ;
#85522=CARTESIAN_POINT ( 'NONE',  ( -67.30776643810303028, -295.1229841594759478, -336.9640344876455060 ) ) ;
#85523=CARTESIAN_POINT ( 'NONE',  ( 17.25982963123163216, -293.8885137752931769, -216.4331697621240380 ) ) ;
#85524=CARTESIAN_POINT ( 'NONE',  ( -71.44909830719414856, -284.1666494155278428, -335.0185077991605453 ) ) ;
#85525=CARTESIAN_POINT ( 'NONE',  ( -21.39194517359764092, -273.3106466430626824, -195.2716677969644365 ) ) ;
#85526=CARTESIAN_POINT ( 'NONE',  ( -40.32648608736790408, -289.7401286725425393, -347.2143011431266473 ) ) ;
#85527=CARTESIAN_POINT ( 'NONE',  ( -110.3083884012011282, -282.4319497071741694, -290.7613112288343018 ) ) ;
#85528=CARTESIAN_POINT ( 'NONE',  ( 21.19297770640138268, -288.4980240389705841, -314.0372790511082144 ) ) ;
#85531=CARTESIAN_POINT ( 'NONE',  ( 179.3481683450128799, 251.2162237358350296, -164.2031354143598492 ) ) ;
#85532=CARTESIAN_POINT ( 'NONE',  ( -37.30987171927208834, -283.5523547857346784, -195.3611179825600175 ) ) ;
#85534=CARTESIAN_POINT ( 'NONE',  ( -98.24276597247360598, -278.0379758613937611, -229.4630841282810536 ) ) ;
#85535=CARTESIAN_POINT ( 'NONE',  ( 39.11606743151551768, -275.3363193404978233, -279.7495316287636911 ) ) ;
#85536=CARTESIAN_POINT ( 'NONE',  ( -109.9447275254303094, -280.3182582703445860, -288.5475079289647624 ) ) ;
#85537=CARTESIAN_POINT ( 'NONE',  ( 27.23156886404066057, -24.64972949587738782, -342.7637830639515073 ) ) ;
#85538=CARTESIAN_POINT ( 'NONE',  ( 22.42587235992054318, -279.4844028041153479, -222.7331297969963089 ) ) ;
#85539=CARTESIAN_POINT ( 'NONE',  ( -100.4344906291615729, -282.0320756914086360, -310.3471119873251496 ) ) ;
#85540=CARTESIAN_POINT ( 'NONE',  ( -100.7698843629572139, -297.7536358669563583, -312.2992698669916081 ) ) ;
#85541=CARTESIAN_POINT ( 'NONE',  ( 30.88361845728635302, -293.6956813646223736, -244.2212184902696492 ) ) ;
#85543=CARTESIAN_POINT ( 'NONE',  ( -108.9038523491274759, -289.4569924473643709, -253.5700453439344528 ) ) ;
#85544=CARTESIAN_POINT ( 'NONE',  ( 26.05582569661106973, -275.6281620950620663, -226.8169079915260795 ) ) ;
#85545=CARTESIAN_POINT ( 'NONE',  ( 8.926447763647503919, -298.8139247038343456, -197.3597661904372558 ) ) ;
#85546=EDGE_LOOP ( 'NONE', ( #64362, #68160, #50638, #90523 ) ) ;
#85551=CARTESIAN_POINT ( 'NONE',  ( -57.21013760975414897, -280.8693607649280466, -199.7957492467839131 ) ) ;
#85552=CARTESIAN_POINT ( 'NONE',  ( -33.98279256658350533, -281.8539990600738179, -194.4487227149543855 ) ) ;
#85553=CARTESIAN_POINT ( 'NONE',  ( 35.54251501220352338, -283.2288194300687110, -256.1961503749483313 ) ) ;
#85554=CARTESIAN_POINT ( 'NONE',  ( 28.48924969137261698, -273.5867518456990410, -237.2402213100553467 ) ) ;
#85557=CARTESIAN_POINT ( 'NONE',  ( -109.5814440185550040, -279.0218213547810251, -296.7002583133177041 ) ) ;
#85561=CARTESIAN_POINT ( 'NONE',  ( -55.28555507663003254, -285.2617727398736633, -343.5487184990271317 ) ) ;
#85562=CARTESIAN_POINT ( 'NONE',  ( 30.73206060456390531, -293.1086534307085572, -297.3057385194401263 ) ) ;
#85564=CARTESIAN_POINT ( 'NONE',  ( 20.49075617362565538, -287.5875370793182810, -321.0634918141067828 ) ) ;
#85565=CARTESIAN_POINT ( 'NONE',  ( -110.4181088180543640, -282.9457908777168313, -258.5416320282533889 ) ) ;
#85566=CARTESIAN_POINT ( 'NONE',  ( -100.1024354129055638, -283.6532775940405031, -231.8392706211699590 ) ) ;
#85567=CARTESIAN_POINT ( 'NONE',  ( -48.23192545448974045, -287.4323272021493949, -343.6206156817993929 ) ) ;
#85568=CARTESIAN_POINT ( 'NONE',  ( -38.87808651764148493, -284.2768934544958483, -343.7546692422877754 ) ) ;
#85569=CARTESIAN_POINT ( 'NONE',  ( -21.74517891133420733, -272.2519085594715875, -197.0007119613921418 ) ) ;
#85570=CARTESIAN_POINT ( 'NONE',  ( -113.3522103628082363, -283.0287314509279781, -264.2914591081551521 ) ) ;
#85571=CARTESIAN_POINT ( 'NONE',  ( -98.36594887961382483, -297.9583063311339970, -314.0494907112497458 ) ) ;
#85572=CARTESIAN_POINT ( 'NONE',  ( -36.55832833323467668, -284.0618060758968682, -195.1858001347452785 ) ) ;
#85573=CARTESIAN_POINT ( 'NONE',  ( -109.1202495476264431, -279.6853521515758416, -255.7637111016307756 ) ) ;
#85574=CARTESIAN_POINT ( 'NONE',  ( 15.00377397118206524, -288.7885883970969871, -216.4168896881612341 ) ) ;
#85576=CARTESIAN_POINT ( 'NONE',  ( 5.656338806266730579, -294.5498868644410777, -208.2283340149834601 ) ) ;
#85578=CARTESIAN_POINT ( 'NONE',  ( -111.2615091041748627, -276.3881652025733615, -283.1203342715262465 ) ) ;
#85579=CARTESIAN_POINT ( 'NONE',  ( -96.44809116857096853, -290.4111250448988244, -221.2429945923644539 ) ) ;
#85580=CARTESIAN_POINT ( 'NONE',  ( -41.10012181139206433, -293.5000739352133223, -344.0780607851497734 ) ) ;
#85581=CARTESIAN_POINT ( 'NONE',  ( -5.328647024294761891, -279.1673293274318439, -204.2066932574586531 ) ) ;
#85582=CARTESIAN_POINT ( 'NONE',  ( -94.87606294870063550, -271.2884047939998595, -223.1065532404639100 ) ) ;
#85583=CARTESIAN_POINT ( 'NONE',  ( -72.88000697145282913, -292.8864205847268636, -205.9745207508094325 ) ) ;
#85584=CARTESIAN_POINT ( 'NONE',  ( -4.829096099716510437, -282.9805209788416391, -202.7746430608542312 ) ) ;
#85585=CARTESIAN_POINT ( 'NONE',  ( -82.54414621805294416, -295.9274207310341467, -208.8182747641742196 ) ) ;
#85586=CARTESIAN_POINT ( 'NONE',  ( 14.66139311657559574, -289.9049298967311756, -322.7263612970771760 ) ) ;
#85587=CARTESIAN_POINT ( 'NONE',  ( -30.76236949919573505, -290.3739616631476679, -194.6077566276133837 ) ) ;
#85588=CARTESIAN_POINT ( 'NONE',  ( -90.25248934431769499, -292.7105322276314610, -219.2159979661156228 ) ) ;
#85590=CARTESIAN_POINT ( 'NONE',  ( -110.5296002037081848, -291.3799112639683244, -268.4677586668598224 ) ) ;
#85592=CARTESIAN_POINT ( 'NONE',  ( -88.39632076739410138, -292.5601965001120561, -213.2521482057046001 ) ) ;
#85593=CARTESIAN_POINT ( 'NONE',  ( 27.87594980850826687, -279.0706561490188164, -232.6110856996642724 ) ) ;
#85594=CARTESIAN_POINT ( 'NONE',  ( -2.439435508157327792, -292.5275188815695060, -206.2311530372823540 ) ) ;
#85595=CARTESIAN_POINT ( 'NONE',  ( 37.98466697166355743, -281.3516765318192938, -254.3312487121299341 ) ) ;
#85596=CARTESIAN_POINT ( 'NONE',  ( 38.23473724657374362, -281.0358927337142063, -255.7342110862453239 ) ) ;
#85597=CARTESIAN_POINT ( 'NONE',  ( 36.48606533473977720, -285.7215866681849548, -283.5695129448341731 ) ) ;
#85598=CARTESIAN_POINT ( 'NONE',  ( 34.31195114662135381, -279.4390737884366445, -250.9057321558088631 ) ) ;
#85599=CARTESIAN_POINT ( 'NONE',  ( -108.0821718506374367, -282.8746962257821451, -245.4455343434404995 ) ) ;
#85601=CARTESIAN_POINT ( 'NONE',  ( -42.36490753274321719, -278.4697658415672663, -194.2199652434757411 ) ) ;
#85602=CARTESIAN_POINT ( 'NONE',  ( -10.09088630242400164, -285.3199135600573300, -198.6185194870605812 ) ) ;
#85603=CARTESIAN_POINT ( 'NONE',  ( 11.64707871944216144, -275.5554826588801234, -215.9541481952816184 ) ) ;
#85605=CARTESIAN_POINT ( 'NONE',  ( 34.55941910400228778, -295.3699824761300761, -287.0502434905782252 ) ) ;
#85606=CARTESIAN_POINT ( 'NONE',  ( 39.11797753642464670, -276.9873318526389312, -271.1473252018745370 ) ) ;
#85607=CARTESIAN_POINT ( 'NONE',  ( -21.65261428490309115, -276.5122992219743878, -341.7289018854619371 ) ) ;
#85608=CARTESIAN_POINT ( 'NONE',  ( -114.0070502354968625, -290.8154066162862250, -262.6390699424250101 ) ) ;
#85610=CARTESIAN_POINT ( 'NONE',  ( 38.08990486678211340, -279.6985883279926952, -275.5861483506444074 ) ) ;
#85611=CARTESIAN_POINT ( 'NONE',  ( -64.38681532129820084, -291.5422200893734725, -198.2108282642895460 ) ) ;
#85612=CARTESIAN_POINT ( 'NONE',  ( -14.76250794572301750, -291.4107899595201729, -200.6934172302254069 ) ) ;
#85613=CARTESIAN_POINT ( 'NONE',  ( -36.32772128997841321, -293.0393184440316077, -345.3670314085981659 ) ) ;
#85616=CARTESIAN_POINT ( 'NONE',  ( -62.81631593080187770, -291.2190038226141837, -201.8846082046662218 ) ) ;
#85618=CARTESIAN_POINT ( 'NONE',  ( -37.37352853689063181, -274.5523547857346784, -340.3611179825599606 ) ) ;
#85619=CARTESIAN_POINT ( 'NONE',  ( -101.3468667017618543, -296.1703763394959878, -227.9560730383263092 ) ) ;
#85620=CARTESIAN_POINT ( 'NONE',  ( -113.8477035252685425, -285.8718581595813930, -270.0009574507120078 ) ) ;
#85621=CARTESIAN_POINT ( 'NONE',  ( 15.03097391921307668, -286.6502169098480977, -219.5073765505128733 ) ) ;
#85622=CARTESIAN_POINT ( 'NONE',  ( -8.449172227651917666, -278.1870730336481188, -338.1680766581016542 ) ) ;
#85623=CARTESIAN_POINT ( 'NONE',  ( -101.5948613704433257, -294.0605653771070251, -308.4547664474541762 ) ) ;
#85624=CARTESIAN_POINT ( 'NONE',  ( -99.57335025802424866, -297.7642799903013042, -310.5198579874615916 ) ) ;
#85625=CARTESIAN_POINT ( 'NONE',  ( -9.853820414761541358, -275.4799099457689522, -338.4302259340467458 ) ) ;
#85628=CARTESIAN_POINT ( 'NONE',  ( -74.59984961037540074, -295.2002672339990568, -337.7823373737829229 ) ) ;
#85629=CARTESIAN_POINT ( 'NONE',  ( 35.10623275568143242, -289.2503028145857229, -253.2002213704480766 ) ) ;
#85630=CARTESIAN_POINT ( 'NONE',  ( -66.71072642002270925, -295.6672788974004789, -201.3367497637570125 ) ) ;
#85631=CARTESIAN_POINT ( 'NONE',  ( -56.08373206472055017, -289.9512813307704278, -341.0722842075379617 ) ) ;
#85633=CARTESIAN_POINT ( 'NONE',  ( -31.08095794509638310, -279.1880403954928056, -193.7996129039383391 ) ) ;
#85634=CARTESIAN_POINT ( 'NONE',  ( -111.1152470976926736, -296.9305095436812962, -292.1049314110994146 ) ) ;
#85635=CARTESIAN_POINT ( 'NONE',  ( -104.8919272473247730, -289.1420248176779637, -235.9341082319315603 ) ) ;
#85636=CARTESIAN_POINT ( 'NONE',  ( -72.06069974033017900, -295.8319812882730844, -339.0658147474513839 ) ) ;
#85637=CARTESIAN_POINT ( 'NONE',  ( -1.249916577458247025, -292.8783556283502776, -206.8685273923465218 ) ) ;
#85640=CARTESIAN_POINT ( 'NONE',  ( -70.32172481685874743, -290.9989759546916730, -339.1869951918496895 ) ) ;
#85641=CARTESIAN_POINT ( 'NONE',  ( -88.47809603358389552, -294.9094976428775681, -206.1857440867352693 ) ) ;
#85643=CARTESIAN_POINT ( 'NONE',  ( 29.20253095018268752, -280.3989211745574721, -231.8231095163028499 ) ) ;
#85644=CARTESIAN_POINT ( 'NONE',  ( -68.52569315994661281, -285.4630320055049424, -338.3874879343434827 ) ) ;
#85645=CARTESIAN_POINT ( 'NONE',  ( -18.31109446836311960, -284.8673060323918662, -196.3034452094861422 ) ) ;
#85646=CARTESIAN_POINT ( 'NONE',  ( -74.28035954010299236, -287.6270583448797424, -335.0043673302799903 ) ) ;
#85647=CARTESIAN_POINT ( 'NONE',  ( 14.06280831804406795, -278.2005351252448691, -326.0911639105086692 ) ) ;
#85649=CARTESIAN_POINT ( 'NONE',  ( -96.88569645718911261, -277.9621966968304037, -312.6144804368162227 ) ) ;
#85650=CARTESIAN_POINT ( 'NONE',  ( 31.16873647268653258, -280.5593790851364702, -244.7165791536186816 ) ) ;
#85651=CARTESIAN_POINT ( 'NONE',  ( 19.79633913834168979, -275.9345203025673072, -219.1290420161784596 ) ) ;
#85652=CARTESIAN_POINT ( 'NONE',  ( -38.15024140828950294, -278.8371609032972742, -193.7624562362642280 ) ) ;
#85653=CARTESIAN_POINT ( 'NONE',  ( 195.2250370176061267, 284.1914500304793023, -110.9006798413472836 ) ) ;
#85654=CARTESIAN_POINT ( 'NONE',  ( -58.06964132618014673, -274.7320905147675489, -196.3925819611789905 ) ) ;
#85655=CARTESIAN_POINT ( 'NONE',  ( -36.21360370459082390, -299.4912800419726295, -193.9500752164755681 ) ) ;
#85657=CARTESIAN_POINT ( 'NONE',  ( -37.30987171927208124, -285.5519495502701943, -345.3611179825600175 ) ) ;
#85659=CARTESIAN_POINT ( 'NONE',  ( 82.62832869962693394, -301.1699953031597943, -193.4454218763038114 ) ) ;
#85660=CARTESIAN_POINT ( 'NONE',  ( 16.24627932075137338, -289.3489404375036997, -320.4609492190604101 ) ) ;
#85661=CARTESIAN_POINT ( 'NONE',  ( -33.79731722162228635, -287.8563145932638463, -194.4571565249364937 ) ) ;
#85662=CARTESIAN_POINT ( 'NONE',  ( 31.07292536875174704, -286.5558212225456032, -244.4629539084911869 ) ) ;
#85663=CARTESIAN_POINT ( 'NONE',  ( -95.76571894798283324, -284.7365381984394048, -220.2196471121708896 ) ) ;
#85664=CARTESIAN_POINT ( 'NONE',  ( -22.00851402745521312, -278.6516009200969961, -198.1191210953321047 ) ) ;
#85665=CARTESIAN_POINT ( 'NONE',  ( 19.59412720405913788, -288.7474324378407005, -222.7054423590212195 ) ) ;
#85666=CARTESIAN_POINT ( 'NONE',  ( 34.31986644239420059, -280.2572973485837338, -287.5998452620785315 ) ) ;
#85667=CARTESIAN_POINT ( 'NONE',  ( -9.788035268694443403, -277.9997528014484374, -338.5072876270148754 ) ) ;
#85668=CARTESIAN_POINT ( 'NONE',  ( -5.286711455162205198, -274.9780947195160365, -204.6931425802561932 ) ) ;
#85669=CARTESIAN_POINT ( 'NONE',  ( -34.69598244527006159, -287.8145275857817182, -346.9183442744681543 ) ) ;
#85670=CARTESIAN_POINT ( 'NONE',  ( -38.71937977508299156, -283.8718481715195594, -347.1872907360625504 ) ) ;
#85671=CARTESIAN_POINT ( 'NONE',  ( -105.3806057996520593, -285.5099239001870046, -234.3271974006147786 ) ) ;
#85672=CARTESIAN_POINT ( 'NONE',  ( 34.70390239981624347, -281.8740417792929520, -282.1267952221280666 ) ) ;
#85676=CARTESIAN_POINT ( 'NONE',  ( -77.46190241506330665, -291.4443009915162293, -334.6926333359923547 ) ) ;
#85677=CARTESIAN_POINT ( 'NONE',  ( -90.43159448846546411, -290.0045755535269336, -215.1989393131665338 ) ) ;
#85678=CARTESIAN_POINT ( 'NONE',  ( -56.91300004569694693, -272.8523595307430014, -199.7364786031569395 ) ) ;
#85680=CARTESIAN_POINT ( 'NONE',  ( 25.62641189995187574, -293.4854557767727670, -314.5239824245462046 ) ) ;
#85681=CARTESIAN_POINT ( 'NONE',  ( -97.13237767597787808, -288.4352696932550089, -313.4399136002857063 ) ) ;
#85682=CARTESIAN_POINT ( 'NONE',  ( 36.65409205586339425, -291.8335557867605417, -273.5547447701430315 ) ) ;
#85683=CARTESIAN_POINT ( 'NONE',  ( 30.32190048286579298, -288.3761207082243345, -241.7907236443691659 ) ) ;
#85684=CARTESIAN_POINT ( 'NONE',  ( -4.771743288812468897, -291.1233781216987495, -337.9199732462171255 ) ) ;
#85685=CARTESIAN_POINT ( 'NONE',  ( -94.84091013533529235, -291.8867198572891084, -318.5353800385944965 ) ) ;
#85686=CARTESIAN_POINT ( 'NONE',  ( -63.72096588275577744, -289.7090353403534664, -199.9204772003336359 ) ) ;
#85687=CARTESIAN_POINT ( 'NONE',  ( -89.77392117723161391, -293.3129983394313172, -216.6623688720681571 ) ) ;
#85688=CARTESIAN_POINT ( 'NONE',  ( -74.85088203869791812, -286.4806232702046032, -207.4606432583150024 ) ) ;
#85689=CARTESIAN_POINT ( 'NONE',  ( 14.16296423689625605, -294.7731795263302388, -215.5420907042164345 ) ) ;
#85690=CARTESIAN_POINT ( 'NONE',  ( -114.2601182895341481, -273.1888302692865977, -270.3692244198358026 ) ) ;
#85692=CARTESIAN_POINT ( 'NONE',  ( 73.72085311440586963, -301.3523753661854130, -194.7650907356766083 ) ) ;
#85693=CARTESIAN_POINT ( 'NONE',  ( -12.90104227253787172, -280.7345018630948061, -341.3221420630307534 ) ) ;
#85694=CARTESIAN_POINT ( 'NONE',  ( -104.4668316174843454, -295.2622832809120723, -307.8647735153213034 ) ) ;
#85695=CARTESIAN_POINT ( 'NONE',  ( -51.73690304907813697, -272.1054623281968929, -197.7086668234656770 ) ) ;
#85696=CARTESIAN_POINT ( 'NONE',  ( -64.88832187261836282, -275.4944709412690145, -339.5714740457713674 ) ) ;
#85697=CARTESIAN_POINT ( 'NONE',  ( -41.91565298661817707, -299.3084846687801246, -197.0104367736587108 ) ) ;
#85698=CARTESIAN_POINT ( 'NONE',  ( 37.06532759786092868, -273.9071475562366800, -252.9202260240812166 ) ) ;
#85700=CARTESIAN_POINT ( 'NONE',  ( -93.52055971136928747, -297.3070798532343701, -317.9128395397153213 ) ) ;
#85702=CARTESIAN_POINT ( 'NONE',  ( -108.1232084552512447, -297.1105650562094525, -288.9195344937976415 ) ) ;
#85704=CARTESIAN_POINT ( 'NONE',  ( 8.823414105639065141, -284.7018156203092190, -210.8028353717432140 ) ) ;
#85705=CARTESIAN_POINT ( 'NONE',  ( -35.14775944149625531, -298.0803702048956438, -197.3611180162293408 ) ) ;
#85706=CARTESIAN_POINT ( 'NONE',  ( -67.18905943793892277, -285.6714749786099219, -199.3812959045337720 ) ) ;
#85707=CARTESIAN_POINT ( 'NONE',  ( 16.66809589160853022, -287.9761739317270894, -325.2867296352273456 ) ) ;
#85708=CARTESIAN_POINT ( 'NONE',  ( -110.6795407128679329, -298.7533848727259169, -253.0415352593796001 ) ) ;
#85709=CARTESIAN_POINT ( 'NONE',  ( -12.42113940956891582, -292.7272644515553566, -340.9776930315268260 ) ) ;
#85710=CARTESIAN_POINT ( 'NONE',  ( -86.69316799550755093, -278.5836415284378518, -211.3970264562993293 ) ) ;
#85711=CARTESIAN_POINT ( 'NONE',  ( -85.33152481854862970, -293.1952119285919593, -330.4860931364851808 ) ) ;
#85713=CARTESIAN_POINT ( 'NONE',  ( 23.06803662453980763, -286.9247910738117184, -312.0701241328527544 ) ) ;
#85715=CARTESIAN_POINT ( 'NONE',  ( -53.87350090601299968, -287.2642022878402486, -343.5164336381164389 ) ) ;
#85716=CARTESIAN_POINT ( 'NONE',  ( -110.2717623132042490, -274.2150852030433725, -259.4328274767220819 ) ) ;
#85717=CARTESIAN_POINT ( 'NONE',  ( 5.836234480685224213, -282.0503584991929529, -207.3192885790292053 ) ) ;
#85718=CARTESIAN_POINT ( 'NONE',  ( -96.98833363688429188, -293.9441976605648961, -316.4120237049493198 ) ) ;
#85719=CARTESIAN_POINT ( 'NONE',  ( 34.48544930250888285, -281.7250038463617443, -283.4642198079997684 ) ) ;
#85720=CARTESIAN_POINT ( 'NONE',  ( -113.6523343058869671, -296.5853779519620730, -281.0319655623688959 ) ) ;
#85721=CARTESIAN_POINT ( 'NONE',  ( -88.62198031439875479, -298.8372975569203049, -217.3649965788345071 ) ) ;
#85722=CARTESIAN_POINT ( 'NONE',  ( 18.61897101117994069, -282.8570347894951738, -220.4078193683573090 ) ) ;
#85723=CARTESIAN_POINT ( 'NONE',  ( -110.4464514635021999, -295.6683673989566614, -265.9903309002061178 ) ) ;
#85726=CARTESIAN_POINT ( 'NONE',  ( -93.78673188038794706, -285.8511835702556709, -319.2252658153869334 ) ) ;
#85728=CARTESIAN_POINT ( 'NONE',  ( 31.98288692825983404, -290.6237833571634042, -237.0123917617631264 ) ) ;
#85729=CARTESIAN_POINT ( 'NONE',  ( 32.86807142883216670, -275.1486438893880404, -301.5820532334019504 ) ) ;
#85730=CARTESIAN_POINT ( 'NONE',  ( -12.25821258863840590, -292.2209570461576504, -201.7520162747607912 ) ) ;
#85731=CARTESIAN_POINT ( 'NONE',  ( 18.47714651961067744, -282.3932482922413669, -222.2276796297211376 ) ) ;
#85732=CARTESIAN_POINT ( 'NONE',  ( -8.406438897629112006, -278.2670665265890193, -338.2658343669842793 ) ) ;
#85733=CARTESIAN_POINT ( 'NONE',  ( -111.3000326655414938, -285.7346250109096673, -289.6163627032206023 ) ) ;
#85734=CARTESIAN_POINT ( 'NONE',  ( 33.50084658414023409, -280.0943080848075510, -251.1175769027694287 ) ) ;
#85735=CARTESIAN_POINT ( 'NONE',  ( -96.00179778450207380, -279.9096711107787883, -317.1148411863597971 ) ) ;
#85736=CARTESIAN_POINT ( 'NONE',  ( -85.80987657102753019, -273.5686025485974824, -210.5293883002286748 ) ) ;
#85737=CARTESIAN_POINT ( 'NONE',  ( 38.49247849006026456, -275.2175914622532105, -256.9374563610105042 ) ) ;
#85738=CARTESIAN_POINT ( 'NONE',  ( 36.64088209824904396, -295.5847777890091379, -279.0549050300811018 ) ) ;
#85742=CARTESIAN_POINT ( 'NONE',  ( -111.4028354867733981, -294.4886743293645281, -286.3377795149082772 ) ) ;
#85743=CARTESIAN_POINT ( 'NONE',  ( 15.63819010738987458, -275.7844356949537996, -320.6713522526613360 ) ) ;
#85744=CARTESIAN_POINT ( 'NONE',  ( 10.77624762452223095, -295.9211792751279972, -329.6522842735044492 ) ) ;
#85745=CARTESIAN_POINT ( 'NONE',  ( 22.86914366386307051, -295.3939904286159503, -317.7389313950892529 ) ) ;
#85746=CARTESIAN_POINT ( 'NONE',  ( 34.85732033990312573, -289.8081786543672820, -290.2343563553295098 ) ) ;
#85747=CARTESIAN_POINT ( 'NONE',  ( -67.56590383719320414, -275.4494358112877990, -338.8193237687033275 ) ) ;
#85748=CARTESIAN_POINT ( 'NONE',  ( -5.641628879685472775, -278.5521394614029873, -337.7281092861886123 ) ) ;
#85749=CARTESIAN_POINT ( 'NONE',  ( -110.1832310492710860, -294.8312661254718137, -254.9563429599116660 ) ) ;
#85750=CARTESIAN_POINT ( 'NONE',  ( 21.57789524123696978, -284.0618348067586112, -318.0133791635034868 ) ) ;
#85751=CARTESIAN_POINT ( 'NONE',  ( -87.89777669145703953, -284.2451970324794956, -217.2733680245724486 ) ) ;
#85752=CARTESIAN_POINT ( 'NONE',  ( 104.9453854588719111, 114.9807708061526768, -282.1350155447395309 ) ) ;
#85754=CARTESIAN_POINT ( 'NONE',  ( -103.0335413260907558, -283.7859501076784454, -302.3625121701737157 ) ) ;
#85755=CARTESIAN_POINT ( 'NONE',  ( 33.28664616673696486, -283.0152322226035153, -300.3820624017549790 ) ) ;
#85756=CARTESIAN_POINT ( 'NONE',  ( -113.7545427575485348, -283.4237204857101347, -264.2644808022508300 ) ) ;
#85757=CARTESIAN_POINT ( 'NONE',  ( -101.7005176884557756, -280.0456748938203759, -228.4227924386562449 ) ) ;
#85758=CARTESIAN_POINT ( 'NONE',  ( -99.07732452895298536, -279.4715437568043512, -315.2321911048433662 ) ) ;
#85759=CARTESIAN_POINT ( 'NONE',  ( -102.0172624299487154, -270.4809262143062369, -239.1787733560258289 ) ) ;
#85760=CARTESIAN_POINT ( 'NONE',  ( -94.53301180112747204, -240.7393305608231913, -341.8848713043685166 ) ) ;
#85762=CARTESIAN_POINT ( 'NONE',  ( -107.1351055028651444, -274.9058821298693260, -243.2197343025253815 ) ) ;
#85763=CARTESIAN_POINT ( 'NONE',  ( -67.95838257802341786, -277.6683635073297864, -202.2702986123385642 ) ) ;
#85764=CARTESIAN_POINT ( 'NONE',  ( -111.0176479060446866, -292.5486748608047947, -251.7121738408289389 ) ) ;
#85765=CARTESIAN_POINT ( 'NONE',  ( 21.89216935441539036, -292.3020215004322040, -227.5001114091085697 ) ) ;
#85766=CARTESIAN_POINT ( 'NONE',  ( -112.8088645201898288, -289.8715453812329201, -285.4023685039321663 ) ) ;
#85768=CARTESIAN_POINT ( 'NONE',  ( 21.81881515393812521, -292.7812609300220856, -318.7411363038077070 ) ) ;
#85769=CARTESIAN_POINT ( 'NONE',  ( -67.86012005591703655, -284.0446007464481681, -203.1668737180935409 ) ) ;
#85770=CARTESIAN_POINT ( 'NONE',  ( -55.33428400204005726, -293.6786350541656816, -198.3393684687820553 ) ) ;
#85771=CARTESIAN_POINT ( 'NONE',  ( -8.283950716791443014, -283.9786676134251593, -337.8658635795046621 ) ) ;
#85773=CARTESIAN_POINT ( 'NONE',  ( -112.6962975145030725, -291.6779892833129679, -255.6466024279604881 ) ) ;
#85774=CARTESIAN_POINT ( 'NONE',  ( -6.749370263548423843, -280.9572518169413797, -203.9991546187190750 ) ) ;
#85775=CARTESIAN_POINT ( 'NONE',  ( 37.07060684332193290, -292.5764034922810310, -288.6043414482115850 ) ) ;
#85776=CARTESIAN_POINT ( 'NONE',  ( 37.66954564181710197, -288.5644961872640692, -287.0787069798631705 ) ) ;
#85777=CARTESIAN_POINT ( 'NONE',  ( -113.9461947854349262, -291.1410213015502677, -262.6493668697426074 ) ) ;
#85778=CARTESIAN_POINT ( 'NONE',  ( 35.65519841913559418, -287.7277101066745217, -271.0340273153930752 ) ) ;
#85781=CARTESIAN_POINT ( 'NONE',  ( -33.47381399219635512, -296.8643924128447225, -346.0400358634137774 ) ) ;
#85782=CARTESIAN_POINT ( 'NONE',  ( -65.34579475146988159, -296.3786194635000015, -199.1071049529226400 ) ) ;
#85783=CARTESIAN_POINT ( 'NONE',  ( -85.26824692627361912, -276.7919171746917755, -325.8038811662642047 ) ) ;
#85784=CARTESIAN_POINT ( 'NONE',  ( -26.99857988267562448, -273.6878153121984951, -194.0676702579505104 ) ) ;
#85785=CARTESIAN_POINT ( 'NONE',  ( -100.7730316895313791, -294.5202615458483137, -307.9739570292107373 ) ) ;
#85786=CARTESIAN_POINT ( 'NONE',  ( 35.62087088786995537, -277.1496272757230486, -257.8586944271748962 ) ) ;
#85787=CARTESIAN_POINT ( 'NONE',  ( -52.82550546027108851, -296.0910042078525635, -197.9329270260638509 ) ) ;
#85788=CARTESIAN_POINT ( 'NONE',  ( 12.63642499629979099, -295.5419929105079859, -324.1831632783031978 ) ) ;
#85789=CARTESIAN_POINT ( 'NONE',  ( -80.32495229518906399, -296.7297519182717451, -329.7468579030024785 ) ) ;
#85791=CARTESIAN_POINT ( 'NONE',  ( -106.6936256947451938, -294.1727584114302658, -299.4845382643239873 ) ) ;
#85792=CARTESIAN_POINT ( 'NONE',  ( -112.9113753381214735, -273.5328259274955371, -256.1706220193983086 ) ) ;
#85793=CARTESIAN_POINT ( 'NONE',  ( -50.87751384109608921, -287.8030658880169881, -342.7468645324327667 ) ) ;
#85794=CARTESIAN_POINT ( 'NONE',  ( -111.5657523610991149, -274.6950462632147492, -259.2447671250016015 ) ) ;
#85795=CARTESIAN_POINT ( 'NONE',  ( -36.94634933104565988, -274.5493541400449544, -193.4106304115468902 ) ) ;
#85796=CARTESIAN_POINT ( 'NONE',  ( -98.46759592877810974, -297.4399682125919639, -230.3232402885087708 ) ) ;
#85797=CARTESIAN_POINT ( 'NONE',  ( -31.23279406911437306, -282.1087133302665961, -195.2023754378563183 ) ) ;
#85798=CARTESIAN_POINT ( 'NONE',  ( 39.03569538216176937, -280.3034709773987743, -275.6436429937372168 ) ) ;
#85799=EDGE_CURVE ( 'NONE', #55239, #54554, #70204, .T. ) ;
#85800=CARTESIAN_POINT ( 'NONE',  ( -8.085360970329940500, -282.0275942556496602, -341.5328336744230455 ) ) ;
#85801=CARTESIAN_POINT ( 'NONE',  ( 29.86249072600618248, -274.4143903612652480, -232.8763482313367490 ) ) ;
#85802=CARTESIAN_POINT ( 'NONE',  ( 37.47315155673641840, -279.7692503375686215, -255.8981174442102144 ) ) ;
#85803=CARTESIAN_POINT ( 'NONE',  ( -12.10041799479818181, -278.3795462083166399, -199.5045815458435072 ) ) ;
#85805=CARTESIAN_POINT ( 'NONE',  ( -43.51359144666648149, -272.5475277165089665, -196.9800407331447332 ) ) ;
#85806=CARTESIAN_POINT ( 'NONE',  ( -19.85633632169537321, -276.2769523627447938, -197.3750361555509585 ) ) ;
#85809=CARTESIAN_POINT ( 'NONE',  ( 19.16243952856850186, -290.8822657840449892, -220.4849307037962944 ) ) ;
#85810=CARTESIAN_POINT ( 'NONE',  ( -47.74339216224365146, -291.9235117316364381, -194.0131243149929503 ) ) ;
#85811=CARTESIAN_POINT ( 'NONE',  ( -12.44871337131436206, -278.7294596728138458, -341.3408056513137012 ) ) ;
#85812=CARTESIAN_POINT ( 'NONE',  ( 22.28671310206897616, -272.9291108996798130, -224.8487290386991333 ) ) ;
#85815=CARTESIAN_POINT ( 'NONE',  ( -102.4604238925557951, -283.0494305424492154, -233.0481712420753695 ) ) ;
#85817=CARTESIAN_POINT ( 'NONE',  ( 30.94940323027170592, -292.7064750406875078, -297.3972325438379585 ) ) ;
#85818=CARTESIAN_POINT ( 'NONE',  ( 17.82413611787097452, -284.9921599658878222, -220.6672302870377109 ) ) ;
#85821=CARTESIAN_POINT ( 'NONE',  ( 2.614354125536130002, -292.5166364664996763, -333.8931922374497390 ) ) ;
#85822=CARTESIAN_POINT ( 'NONE',  ( -44.37476865659339609, -281.6193288297670279, -346.3958598503389226 ) ) ;
#85823=CARTESIAN_POINT ( 'NONE',  ( -105.1854217436183063, -280.5382327403985983, -241.3151225513428813 ) ) ;
#85824=CARTESIAN_POINT ( 'NONE',  ( -103.7041802232159426, -286.2583951535875713, -231.9929530054473048 ) ) ;
#85825=CARTESIAN_POINT ( 'NONE',  ( 24.27231187649644184, -280.3898207318718505, -314.8543957327372596 ) ) ;
#85826=CARTESIAN_POINT ( 'NONE',  ( 2.447014477759043238, -286.6019865148135182, -209.1577014928330414 ) ) ;
#85827=CARTESIAN_POINT ( 'NONE',  ( -40.51313852930374537, -278.5180517248779779, -343.8945433916259162 ) ) ;
#85828=CARTESIAN_POINT ( 'NONE',  ( -80.90735955920331435, -278.4638174307096392, -329.1372614830498264 ) ) ;
#85829=CARTESIAN_POINT ( 'NONE',  ( -82.31488457452613261, -287.4221278830089545, -209.8326594777478533 ) ) ;
#85831=CARTESIAN_POINT ( 'NONE',  ( 30.79044743357041725, -298.7164300005194377, -193.3629520540350768 ) ) ;
#85832=CARTESIAN_POINT ( 'NONE',  ( 13.28957391886754635, -290.3202489952476526, -325.2795396473097185 ) ) ;
#85834=CARTESIAN_POINT ( 'NONE',  ( -88.52914483777347243, -275.9090924074130271, -206.2264541496106460 ) ) ;
#85836=CARTESIAN_POINT ( 'NONE',  ( 23.84961573162311055, -272.9594273835972444, -226.6853232383336945 ) ) ;
#85837=CARTESIAN_POINT ( 'NONE',  ( 37.28265016409321930, -291.7564006316505925, -254.8812888575445754 ) ) ;
#85838=CARTESIAN_POINT ( 'NONE',  ( -93.99423961548697548, -295.4071145937429037, -316.5162158226945053 ) ) ;
#85839=CARTESIAN_POINT ( 'NONE',  ( 28.26667228697986900, -288.6192598304143075, -236.6890277552311659 ) ) ;
#85840=CARTESIAN_POINT ( 'NONE',  ( -1.494647797404490053, -282.2945127053787928, -205.6080265215061331 ) ) ;
#85841=CARTESIAN_POINT ( 'NONE',  ( -12.39878815453698024, -290.1593695883699411, -342.6416145997918079 ) ) ;
#85842=CARTESIAN_POINT ( 'NONE',  ( -54.37541671862952342, -290.5815790275290169, -345.0020090174414804 ) ) ;
#85843=CARTESIAN_POINT ( 'NONE',  ( -88.26870779457259175, -285.7650690485356790, -325.4906657391997555 ) ) ;
#85844=CARTESIAN_POINT ( 'NONE',  ( -114.0789197055876656, -278.6316363909194820, -277.3331901124690262 ) ) ;
#85845=CARTESIAN_POINT ( 'NONE',  ( 20.25385196770011476, -292.3038888789243970, -319.2698756806485676 ) ) ;
#85846=CARTESIAN_POINT ( 'NONE',  ( 35.32839188608864589, -281.0625917986267837, -244.7448771800976886 ) ) ;
#85847=CARTESIAN_POINT ( 'NONE',  ( -74.91874138816510253, -275.4069004883340313, -206.2794439007923017 ) ) ;
#85848=CARTESIAN_POINT ( 'NONE',  ( -4.771743288812468897, -291.1233781216987495, -337.9199732462171255 ) ) ;
#85849=CARTESIAN_POINT ( 'NONE',  ( 32.78710686273940667, -273.4134517781415070, -240.9689351963718025 ) ) ;
#85851=CARTESIAN_POINT ( 'NONE',  ( 26.51566355916656192, -280.5748518290793072, -234.8614624291071493 ) ) ;
#85852=CARTESIAN_POINT ( 'NONE',  ( -48.42130949917548577, -278.3951211357284592, -346.2121669165729259 ) ) ;
#85853=CARTESIAN_POINT ( 'NONE',  ( -34.46908655563495927, -299.5140766823485023, -196.7711715412838203 ) ) ;
#85854=CARTESIAN_POINT ( 'NONE',  ( -69.68275518038723249, -284.6954935745990269, -200.7272858806688021 ) ) ;
#85855=CARTESIAN_POINT ( 'NONE',  ( -108.7351969225418884, -292.5666290335522604, -250.8433663041809609 ) ) ;
#85856=CARTESIAN_POINT ( 'NONE',  ( -83.11596427144279176, -275.0376802593943921, -209.3757974498577141 ) ) ;
#85858=CARTESIAN_POINT ( 'NONE',  ( -49.65647411403506339, -275.2135604399873614, -194.7984205639671700 ) ) ;
#85859=FACE_OUTER_BOUND ( 'NONE', #42579, .T. ) ;
#85861=CARTESIAN_POINT ( 'NONE',  ( -28.65858273116080568, -296.9420813793094567, -344.7412818163851398 ) ) ;
#85862=CARTESIAN_POINT ( 'NONE',  ( -36.19024188133170838, -281.0375223410755439, -345.1855964259405027 ) ) ;
#85863=CARTESIAN_POINT ( 'NONE',  ( -98.32890813025441901, -290.8460570862450254, -223.3684722317218814 ) ) ;
#85864=CARTESIAN_POINT ( 'NONE',  ( 37.24410522536589241, -273.6247056781155038, -274.4268006788329330 ) ) ;
#85865=CARTESIAN_POINT ( 'NONE',  ( -43.62087830060645643, -287.5743322721689310, -194.3675640441131520 ) ) ;
#85866=CARTESIAN_POINT ( 'NONE',  ( -62.89565014937137732, -290.6317743444828920, -201.6499710564887096 ) ) ;
#85868=CARTESIAN_POINT ( 'NONE',  ( -112.3430818000429099, -289.3118475998882104, -255.6848548715323659 ) ) ;
#85869=CARTESIAN_POINT ( 'NONE',  ( -83.83923711355822661, -291.0595442950219649, -214.0577740235804072 ) ) ;
#85871=CARTESIAN_POINT ( 'NONE',  ( 20.34948352732071797, -289.3183420156282750, -320.9103019499520428 ) ) ;
#85872=CARTESIAN_POINT ( 'NONE',  ( 15.61613512433503459, -276.6099308755381116, -320.6359145724442783 ) ) ;
#85873=CARTESIAN_POINT ( 'NONE',  ( -5.936905153447610495, -293.5692387928554581, -340.3270480010504002 ) ) ;
#85874=CARTESIAN_POINT ( 'NONE',  ( -113.8016262650160115, -285.1009116203874214, -278.5582200044751744 ) ) ;
#85875=CARTESIAN_POINT ( 'NONE',  ( -89.87491651513268209, -285.6682064388401727, -214.0213469282071230 ) ) ;
#85876=CARTESIAN_POINT ( 'NONE',  ( 33.96197988333747020, -282.0930632603577806, -286.1050915504005729 ) ) ;
#85877=CARTESIAN_POINT ( 'NONE',  ( -39.76822214190186600, -139.5689616928363250, -364.7666786286931710 ) ) ;
#85878=CARTESIAN_POINT ( 'NONE',  ( 192.6862340675979794, 279.0923067692335167, -125.4747399153907423 ) ) ;
#85879=CARTESIAN_POINT ( 'NONE',  ( -110.9460938673244925, -268.0485775136007760, -295.3054752808368448 ) ) ;
#85880=CARTESIAN_POINT ( 'NONE',  ( -56.89495719884656211, -272.9907566640177379, -199.8081319336176023 ) ) ;
#85881=CARTESIAN_POINT ( 'NONE',  ( 32.35998771573641619, -274.1704188865296032, -247.4842727566924623 ) ) ;
#85882=CARTESIAN_POINT ( 'NONE',  ( -50.46320073889224034, -294.7229112231660224, -346.2263198580622543 ) ) ;
#85883=CARTESIAN_POINT ( 'NONE',  ( -110.4703031237083479, -271.8150658180700816, -270.3517331077227368 ) ) ;
#85884=CARTESIAN_POINT ( 'NONE',  ( -63.37345732133692167, -272.4047490413110495, -198.4191560288155642 ) ) ;
#85885=CARTESIAN_POINT ( 'NONE',  ( -86.94290714680967369, -299.2133778354631772, -215.1290101081950183 ) ) ;
#85886=CARTESIAN_POINT ( 'NONE',  ( -50.82562026649912212, -290.5430711862491648, -342.6587482699363250 ) ) ;
#85887=CARTESIAN_POINT ( 'NONE',  ( -67.94270306975059270, -292.7204072126145888, -203.7304741619769572 ) ) ;
#85889=CARTESIAN_POINT ( 'NONE',  ( -101.3601039914526183, -298.0525766679422190, -227.9760602943774188 ) ) ;
#85890=CARTESIAN_POINT ( 'NONE',  ( 19.56536138227702182, -288.6917730722765896, -316.1822352991061393 ) ) ;
#85891=CARTESIAN_POINT ( 'NONE',  ( 15.37534463307258292, -295.1324017058364007, -326.2634615092802619 ) ) ;
#85892=CARTESIAN_POINT ( 'NONE',  ( -70.77545756792481768, -295.9736512146345717, -339.6699936239069757 ) ) ;
#85893=CARTESIAN_POINT ( 'NONE',  ( 23.34006628128329197, -293.1552800687647959, -229.7812802556142344 ) ) ;
#85894=ORIENTED_EDGE ( 'NONE', *, *, #33593, .F. ) ;
#85895=CARTESIAN_POINT ( 'NONE',  ( 33.36547123559886074, -277.1288044683890348, -243.7188561796357646 ) ) ;
#85897=CARTESIAN_POINT ( 'NONE',  ( -88.88556909322818456, -278.8583153894616657, -213.2405746099364876 ) ) ;
#85899=CARTESIAN_POINT ( 'NONE',  ( 36.38736679794425299, -273.8965842165549134, -266.1130124511934127 ) ) ;
#85900=CARTESIAN_POINT ( 'NONE',  ( 21.66366780981341833, -275.8875566233835457, -226.9816873368371546 ) ) ;
#85901=CARTESIAN_POINT ( 'NONE',  ( -13.40324992060266496, -276.1189731458235883, -198.2436817139098082 ) ) ;
#85902=CARTESIAN_POINT ( 'NONE',  ( 37.73949906315206704, -273.6543057514366524, -276.7814239591461387 ) ) ;
#85903=CARTESIAN_POINT ( 'NONE',  ( -39.17919470572959995, -298.6799372295545822, -197.2698558067367003 ) ) ;
#85904=CARTESIAN_POINT ( 'NONE',  ( -110.9633506204263540, -295.1485881538445710, -268.7016428887591246 ) ) ;
#85906=CARTESIAN_POINT ( 'NONE',  ( -79.88198220455588228, -279.9861425904303474, -206.1890838177548915 ) ) ;
#85907=CARTESIAN_POINT ( 'NONE',  ( 16.53258862093414905, -276.4256463369239896, -319.6398988981445655 ) ) ;
#85908=CARTESIAN_POINT ( 'NONE',  ( 0.05744414204401958324, -285.2239752474326906, -203.6033582223108169 ) ) ;
#85909=CARTESIAN_POINT ( 'NONE',  ( -102.5048116201718926, -275.0486224183449622, -233.1250473379532480 ) ) ;
#85910=CARTESIAN_POINT ( 'NONE',  ( 82.65035235331711760, -299.4402615872036790, -197.8644493715226531 ) ) ;
#85911=CARTESIAN_POINT ( 'NONE',  ( 22.87701180632885922, -287.3269692967478477, -311.9320644950454380 ) ) ;
#85912=CARTESIAN_POINT ( 'NONE',  ( -66.44783850786315327, -277.9055762000330105, -202.2972607502154858 ) ) ;
#85913=CARTESIAN_POINT ( 'NONE',  ( -35.63105069429413874, -278.6487229050646306, -196.7792698591719613 ) ) ;
#85915=CARTESIAN_POINT ( 'NONE',  ( -35.15257581845639834, -285.0248523139926533, -345.3418173332767651 ) ) ;
#85916=CARTESIAN_POINT ( 'NONE',  ( -6.093714602630924126, -277.8371768665330706, -336.7880182516466334 ) ) ;
#85918=CARTESIAN_POINT ( 'NONE',  ( -17.64248802589491660, -275.0412929209162485, -343.7499117727878684 ) ) ;
#85919=CARTESIAN_POINT ( 'NONE',  ( 31.21103360533861348, -275.8655311557355958, -244.9757803702410115 ) ) ;
#85920=CARTESIAN_POINT ( 'NONE',  ( 37.58221360234861663, -283.4749831303787460, -264.3249291374853556 ) ) ;
#85922=CARTESIAN_POINT ( 'NONE',  ( 32.71655054365363924, -289.8400890457534729, -298.8052886702989213 ) ) ;
#85923=CARTESIAN_POINT ( 'NONE',  ( 22.69887783722546004, -292.1662705975508061, -315.3280756122244384 ) ) ;
#85926=CARTESIAN_POINT ( 'NONE',  ( -54.30924655656728817, -272.5144278092167838, -198.8534551430940382 ) ) ;
#85927=CARTESIAN_POINT ( 'NONE',  ( -9.238263802550241266, -290.5629460370223569, -201.5964267825922036 ) ) ;
#85928=CARTESIAN_POINT ( 'NONE',  ( 173.4479467868932829, 229.7134184023448142, -192.0138545908111496 ) ) ;
#85930=CARTESIAN_POINT ( 'NONE',  ( -94.94772175729167429, -288.3495179891542080, -320.4036401610202347 ) ) ;
#85931=CARTESIAN_POINT ( 'NONE',  ( -66.86105440172073600, -285.0456632616154593, -338.0139378429362864 ) ) ;
#85932=CARTESIAN_POINT ( 'NONE',  ( 34.89284013776482851, -285.4894424775635002, -246.6099580098289437 ) ) ;
#85933=CARTESIAN_POINT ( 'NONE',  ( -37.52390010888706939, -284.4797863188920815, -343.9626527703907755 ) ) ;
#85934=CARTESIAN_POINT ( 'NONE',  ( -66.61481316073835046, -284.2484963339716728, -337.4245992952517668 ) ) ;
#85935=CARTESIAN_POINT ( 'NONE',  ( -40.58736291348640179, -293.9914421694584235, -195.0629435506246523 ) ) ;
#85936=CARTESIAN_POINT ( 'NONE',  ( -9.760655200936342979, -274.7745141898054158, -340.7074054403451555 ) ) ;
#85937=CARTESIAN_POINT ( 'NONE',  ( -78.83372969306191180, -273.8424907381246953, -205.5216564328746642 ) ) ;
#85938=CARTESIAN_POINT ( 'NONE',  ( -97.03727617580648257, -288.0016320758110169, -316.6833847914109015 ) ) ;
#85939=CARTESIAN_POINT ( 'NONE',  ( 5.871282177220538578, -276.4837123355122799, -334.0921007168759047 ) ) ;
#85940=CARTESIAN_POINT ( 'NONE',  ( 15.49803347003856935, -296.2809052283840288, -323.1577176977123145 ) ) ;
#85943=CARTESIAN_POINT ( 'NONE',  ( -110.0980856356287774, -283.3729883903341147, -259.9807593171267399 ) ) ;
#85944=CARTESIAN_POINT ( 'NONE',  ( -5.762308662806248982, -278.4672254764807917, -202.3336037881050231 ) ) ;
#85945=CARTESIAN_POINT ( 'NONE',  ( -57.91589512562487130, -272.2711127407536083, -196.8255166606715818 ) ) ;
#85947=CARTESIAN_POINT ( 'NONE',  ( -68.08783551814624957, -276.8154440312503084, -336.6965851554475648 ) ) ;
#85948=CARTESIAN_POINT ( 'NONE',  ( 9.272577327340115971, -294.2258041345485822, -213.2176548307470512 ) ) ;
#85949=CARTESIAN_POINT ( 'NONE',  ( 35.94350546125161827, -294.4985136184255907, -270.7492459827872153 ) ) ;
#85950=CARTESIAN_POINT ( 'NONE',  ( -39.07974089614672408, -296.3887040484181625, -346.8482246648846399 ) ) ;
#85951=CARTESIAN_POINT ( 'NONE',  ( -110.3841501660415929, -296.3709617512534464, -271.4609986234810322 ) ) ;
#85952=CARTESIAN_POINT ( 'NONE',  ( -20.66039113737006616, -290.8381335202012110, -343.4824867879971748 ) ) ;
#85953=CARTESIAN_POINT ( 'NONE',  ( -10.70004235915474489, -282.8809172882288294, -342.6619485668637139 ) ) ;
#85954=CARTESIAN_POINT ( 'NONE',  ( 0.5977476434719330989, -272.6917782151280676, -204.7647994963298572 ) ) ;
#85955=CARTESIAN_POINT ( 'NONE',  ( -0.9676835456519505829, -286.3547910630731508, -202.4941088972821035 ) ) ;
#85956=CARTESIAN_POINT ( 'NONE',  ( -74.81773544421018585, -279.5336424865202503, -334.9164708208372190 ) ) ;
#85957=CARTESIAN_POINT ( 'NONE',  ( -74.83029263721171276, -284.5984229527799130, -207.4483698322567875 ) ) ;
#85959=CARTESIAN_POINT ( 'NONE',  ( -26.46055136010997799, -286.9135113292617802, -344.5675951129986174 ) ) ;
#85960=CARTESIAN_POINT ( 'NONE',  ( 2.709286185474054420, -58.23210827017373248, -348.3322198635470954 ) ) ;
#85961=CARTESIAN_POINT ( 'NONE',  ( 33.77165796281082777, -286.8381924516382355, -253.5475924985559573 ) ) ;
#85962=CARTESIAN_POINT ( 'NONE',  ( 9.076082880525564889, -283.3735003560506129, -331.5020178193938705 ) ) ;
#85963=CARTESIAN_POINT ( 'NONE',  ( -113.4312682712157851, -289.7432163818066329, -259.8137745753052741 ) ) ;
#85964=CARTESIAN_POINT ( 'NONE',  ( -113.5841242182532227, -280.1364241277045153, -271.6157743956738386 ) ) ;
#85965=ADVANCED_FACE ( 'NONE', ( #35573 ), #74779, .F. ) ;
#85966=CARTESIAN_POINT ( 'NONE',  ( -98.19436196449558452, -280.4896675398520074, -223.9689636621413911 ) ) ;
#85967=CARTESIAN_POINT ( 'NONE',  ( 4.924881791221928040, -280.4747136745269813, -210.8419105168581495 ) ) ;
#85968=CARTESIAN_POINT ( 'NONE',  ( -8.217062978642150739, -276.4335520214409598, -201.1916585937143509 ) ) ;
#85969=CARTESIAN_POINT ( 'NONE',  ( -37.68897832448769236, -295.0563522512570103, -347.3734132593388608 ) ) ;
#85970=CARTESIAN_POINT ( 'NONE',  ( -89.83528364984188386, -287.8177202881306584, -323.4296631904845754 ) ) ;
#85971=CARTESIAN_POINT ( 'NONE',  ( -16.86142019535844128, -293.9124984013223525, -196.9649426907715508 ) ) ;
#85972=CARTESIAN_POINT ( 'NONE',  ( -99.00071117008862132, -294.9249251930083915, -310.1075418388273306 ) ) ;
#85974=CARTESIAN_POINT ( 'NONE',  ( -53.98836308670775708, -285.1875367435472413, -342.9690516050077349 ) ) ;
#85975=CARTESIAN_POINT ( 'NONE',  ( -102.5493050419904790, -296.6661474953726838, -237.3843446948425253 ) ) ;
#85976=CARTESIAN_POINT ( 'NONE',  ( 35.98737601237200323, -294.3486912546890721, -247.9036225248621577 ) ) ;
#85977=CARTESIAN_POINT ( 'NONE',  ( 21.40594965552208606, -281.5941909678725779, -226.8359576003650204 ) ) ;
#85978=CARTESIAN_POINT ( 'NONE',  ( 23.45386207502789944, -273.9832646113330838, -223.4705401649432019 ) ) ;
#85979=CARTESIAN_POINT ( 'NONE',  ( -36.08018398855008968, -289.6881677601465412, -347.2619300671955216 ) ) ;
#85980=CARTESIAN_POINT ( 'NONE',  ( -2.227978823967796007, -280.7319879563972336, -337.4977850064483960 ) ) ;
#85981=CARTESIAN_POINT ( 'NONE',  ( -111.6135164223091749, -291.1394980910995969, -250.0764264207907956 ) ) ;
#85982=CARTESIAN_POINT ( 'NONE',  ( 10.13222925168583544, -288.7098445959157402, -325.9105300489302408 ) ) ;
#85985=CARTESIAN_POINT ( 'NONE',  ( -21.69536100719032845, -108.9780876184144347, -358.8618341835472734 ) ) ;
#85986=CARTESIAN_POINT ( 'NONE',  ( -112.3381139276884824, -270.1608578419545097, -261.8788190812425114 ) ) ;
#85987=CARTESIAN_POINT ( 'NONE',  ( -100.9471620744349849, -278.2433594110846116, -234.2093969009453645 ) ) ;
#85989=CARTESIAN_POINT ( 'NONE',  ( -38.34432427491105955, -278.9596227473332419, -197.0464084888813829 ) ) ;
#85990=CARTESIAN_POINT ( 'NONE',  ( 31.23338553702003750, -274.7683186972061549, -235.3868143088527063 ) ) ;
#85991=CARTESIAN_POINT ( 'NONE',  ( 66.61766131416349879, 45.94256429874008063, -316.6294464272367577 ) ) ;
#85992=CARTESIAN_POINT ( 'NONE',  ( -64.51567692195030190, -278.2791486848208251, -198.8897714850879765 ) ) ;
#85993=CARTESIAN_POINT ( 'NONE',  ( -15.67870750511635158, -280.7905655471012665, -341.7933344608741209 ) ) ;
#85994=CARTESIAN_POINT ( 'NONE',  ( -106.2380411386437089, -297.8965983094840340, -302.4121430309786547 ) ) ;
#85996=CARTESIAN_POINT ( 'NONE',  ( 27.53831140029111779, -293.5880281851692075, -236.7668841686492556 ) ) ;
#85998=CARTESIAN_POINT ( 'NONE',  ( -110.1866357209424905, -289.3695290652068479, -260.2447464865329039 ) ) ;
#85999=CARTESIAN_POINT ( 'NONE',  ( 39.21499083192103541, -276.1061511060821658, -262.5823958574994776 ) ) ;
#86000=CARTESIAN_POINT ( 'NONE',  ( -59.47564202369844111, -273.7575572872853513, -200.7446383398520311 ) ) ;
#86005=CARTESIAN_POINT ( 'NONE',  ( -69.88986283944664990, -280.6927530737937673, -204.6597464184988553 ) ) ;
#86006=CARTESIAN_POINT ( 'NONE',  ( 7.924666833472360672, -282.4208943661107583, -209.2635198249893165 ) ) ;
#86007=CARTESIAN_POINT ( 'NONE',  ( -80.77528869267112555, -282.7163288302032242, -329.3897332318655913 ) ) ;
#86008=CARTESIAN_POINT ( 'NONE',  ( -35.65814349349031431, -281.9338796490721393, -196.1323940554310354 ) ) ;
#86009=CARTESIAN_POINT ( 'NONE',  ( 14.20257346326613401, -274.7922469214290118, -323.0999522957188788 ) ) ;
#86012=CARTESIAN_POINT ( 'NONE',  ( -107.4246183105436927, -278.9503056384033925, -301.9952054448382910 ) ) ;
#86016=CARTESIAN_POINT ( 'NONE',  ( -89.28568953398718122, -285.7583477470764137, -325.0241125775010573 ) ) ;
#86017=CARTESIAN_POINT ( 'NONE',  ( 34.99606262804381629, -292.8977476760435366, -281.6379359963180491 ) ) ;
#86018=CARTESIAN_POINT ( 'NONE',  ( 37.72362617664776963, -287.1104858160874187, -287.1098099827382271 ) ) ;
#86019=CARTESIAN_POINT ( 'NONE',  ( -96.56347389551022786, -283.4066579724055828, -225.9679256277046591 ) ) ;
#86020=CARTESIAN_POINT ( 'NONE',  ( -110.4603487888587665, -283.0123786079946058, -279.1105376037121459 ) ) ;
#86021=CARTESIAN_POINT ( 'NONE',  ( 6.426059300490751802, -286.6886229282208660, -330.1104613063091051 ) ) ;
#86023=CARTESIAN_POINT ( 'NONE',  ( 19.67013053928295818, -283.4079134921353216, -316.6062690709638900 ) ) ;
#86024=CARTESIAN_POINT ( 'NONE',  ( -41.06725506839342188, -272.0052366240666970, -195.4027992210114633 ) ) ;
#86025=CARTESIAN_POINT ( 'NONE',  ( -106.2905221562944860, -282.5321262878493940, -302.8033798383515318 ) ) ;
#86026=CARTESIAN_POINT ( 'NONE',  ( -110.3528192457910961, -298.3312968219668164, -287.5740104511055506 ) ) ;
#86027=CARTESIAN_POINT ( 'NONE',  ( -0.5898072669017507819, -284.5390993879458392, -204.7771743594223040 ) ) ;
#86028=CARTESIAN_POINT ( 'NONE',  ( -66.17333680887702485, -280.6065328909930940, -203.0262249094810727 ) ) ;
#86029=CARTESIAN_POINT ( 'NONE',  ( 37.52379666896567301, -289.6384337980255168, -277.0831574094953567 ) ) ;
#86032=CARTESIAN_POINT ( 'NONE',  ( 32.10296191605898741, -295.8603212217515761, -300.2717559984726563 ) ) ;
#86033=CARTESIAN_POINT ( 'NONE',  ( -71.38271542569091821, -275.5015684762772707, -337.1908264198191887 ) ) ;
#86034=CARTESIAN_POINT ( 'NONE',  ( -97.33107391121868091, -290.3938534175048858, -222.3461843208778532 ) ) ;
#86035=CARTESIAN_POINT ( 'NONE',  ( 23.58201381024364807, -292.5263730467446521, -312.1006772726630061 ) ) ;
#86036=CARTESIAN_POINT ( 'NONE',  ( -46.50142708007193448, -278.6184389651788251, -197.3895586899560328 ) ) ;
#86037=CARTESIAN_POINT ( 'NONE',  ( -33.71316256091402153, -296.2376274846301385, -196.1270752847585186 ) ) ;
#86038=CARTESIAN_POINT ( 'NONE',  ( -102.8567301656565860, -292.3179145393797285, -236.9463972831280500 ) ) ;
#86039=CARTESIAN_POINT ( 'NONE',  ( -69.91165696735023971, -276.1233781216988064, -202.8022627189028810 ) ) ;
#86040=CARTESIAN_POINT ( 'NONE',  ( 6.202332008376906458, -292.9531029290223501, -333.0882781293727248 ) ) ;
#86041=CARTESIAN_POINT ( 'NONE',  ( -97.19563393301493193, -291.5550159112387405, -313.5345707563162136 ) ) ;
#86042=CARTESIAN_POINT ( 'NONE',  ( -47.58431480887909260, -290.1636540129537138, -195.0148536498188037 ) ) ;
#86043=CARTESIAN_POINT ( 'NONE',  ( -37.24920246201178031, -290.4762459037178814, -343.9502908503229150 ) ) ;
#86045=CARTESIAN_POINT ( 'NONE',  ( -3.282106225573130587, -289.3934417777558679, -335.1671021484442008 ) ) ;
#86047=CARTESIAN_POINT ( 'NONE',  ( -95.14852368630150181, -291.0742752973205256, -320.6242244272600033 ) ) ;
#86048=CARTESIAN_POINT ( 'NONE',  ( 37.04014140497751839, -279.7275698075816308, -282.5141891068121254 ) ) ;
#86049=CARTESIAN_POINT ( 'NONE',  ( -107.7258078396471177, -290.2940394252267424, -289.9143129309625238 ) ) ;
#86050=CARTESIAN_POINT ( 'NONE',  ( -71.22911091300672126, -279.9502438134891804, -201.2424686760486168 ) ) ;
#86051=CARTESIAN_POINT ( 'NONE',  ( 39.68930748857101065, -281.2135362459235921, -269.9346225428723187 ) ) ;
#86052=CARTESIAN_POINT ( 'NONE',  ( 37.10650904063178501, -285.6685888660213095, -279.4421311190098436 ) ) ;
#86054=CARTESIAN_POINT ( 'NONE',  ( 33.40130573111337497, -279.9870673443629130, -293.0293091108346744 ) ) ;
#86055=CARTESIAN_POINT ( 'NONE',  ( -29.64225779535219019, -284.1495032150146471, -195.7573698474652986 ) ) ;
#86057=CARTESIAN_POINT ( 'NONE',  ( -99.67137328458505863, -277.6198250861004340, -226.3415814388513070 ) ) ;
#86058=CARTESIAN_POINT ( 'NONE',  ( -23.82681155051151123, -285.1411338649730283, -194.8164535336805159 ) ) ;
#86059=CARTESIAN_POINT ( 'NONE',  ( -85.42396705455898598, -274.1704161940028257, -215.1510692774234315 ) ) ;
#86061=CARTESIAN_POINT ( 'NONE',  ( -65.65249300661895404, -293.2757740169525960, -202.1936613908745244 ) ) ;
#86062=CARTESIAN_POINT ( 'NONE',  ( 37.63703529265601588, -276.7918553247759519, -255.6371399502399981 ) ) ;
#86063=CARTESIAN_POINT ( 'NONE',  ( -108.7863419446854465, -278.0198468780952794, -285.4525275443737655 ) ) ;
#86064=CARTESIAN_POINT ( 'NONE',  ( -68.09256332694990022, -297.4560484384575716, -338.7812279068012913 ) ) ;
#86065=CARTESIAN_POINT ( 'NONE',  ( -88.65106368238826917, -291.5219679919231908, -212.9472763053174162 ) ) ;
#86066=CARTESIAN_POINT ( 'NONE',  ( 28.05278311732715579, -279.1303846559010822, -232.5077725953603931 ) ) ;
#86067=CARTESIAN_POINT ( 'NONE',  ( 1.701931895804736472, -292.3921144411266937, -203.9330621178176273 ) ) ;
#86069=CARTESIAN_POINT ( 'NONE',  ( -86.07669835838689210, -290.4157470530197998, -215.6274482700807482 ) ) ;
#86070=CARTESIAN_POINT ( 'NONE',  ( -87.29289316236092588, -293.7478560305256110, -326.3761031373976493 ) ) ;
#86073=CARTESIAN_POINT ( 'NONE',  ( 19.39754396006932069, -292.4089328173803892, -224.3125701546319704 ) ) ;
#86075=CARTESIAN_POINT ( 'NONE',  ( -105.5795714935544112, -276.2666405000204009, -254.7536222014695397 ) ) ;
#86076=CARTESIAN_POINT ( 'NONE',  ( -94.48446673430025555, -294.9131301214216592, -321.6400900069639874 ) ) ;
#86077=CARTESIAN_POINT ( 'NONE',  ( -113.3317776220491169, -285.9790618700961318, -261.4838213963163298 ) ) ;
#86078=CARTESIAN_POINT ( 'NONE',  ( 26.36841721611366296, -286.8967647944322152, -234.6203349706351275 ) ) ;
#86079=CARTESIAN_POINT ( 'NONE',  ( 19.73073150001051701, -277.7263312491641614, -317.0012339431818873 ) ) ;
#86080=CARTESIAN_POINT ( 'NONE',  ( -41.14774837607774316, -293.1203714731076957, -344.9216765362599517 ) ) ;
#86081=CARTESIAN_POINT ( 'NONE',  ( -53.34696732310778344, -297.0202432051246433, -342.6758818495331411 ) ) ;
#86082=CARTESIAN_POINT ( 'NONE',  ( 29.50964426273811725, -274.7532410796671911, -300.6600991005429364 ) ) ;
#86085=CARTESIAN_POINT ( 'NONE',  ( -113.9226162255255588, -296.1210810376899758, -278.1782518018537189 ) ) ;
#86086=CARTESIAN_POINT ( 'NONE',  ( 36.39000885337114255, -289.6060405823153587, -280.6986184847754089 ) ) ;
#86087=CARTESIAN_POINT ( 'NONE',  ( -82.24831055652813916, -295.4397336948744055, -210.2272085308262035 ) ) ;
#86088=CARTESIAN_POINT ( 'NONE',  ( -111.4381795210764636, -274.0040958469344332, -250.7229238802001134 ) ) ;
#86089=ADVANCED_FACE ( 'NONE', ( #64487 ), #42172, .T. ) ;
#86090=CARTESIAN_POINT ( 'NONE',  ( 34.11207735671815300, -288.4076269515787772, -285.8552187274494258 ) ) ;
#86092=CARTESIAN_POINT ( 'NONE',  ( 20.89544887160410624, -279.9336132315721102, -220.3285809885624644 ) ) ;
#86093=CARTESIAN_POINT ( 'NONE',  ( 13.33489418193412135, -295.0166845592861478, -328.2693917963862873 ) ) ;
#86094=CARTESIAN_POINT ( 'NONE',  ( -45.90999735546880345, -287.2991386654720714, -345.6921402247899096 ) ) ;
#86096=CARTESIAN_POINT ( 'NONE',  ( -110.7783481901860512, -296.5948012587943481, -293.4877565563230064 ) ) ;
#86097=CARTESIAN_POINT ( 'NONE',  ( 24.44741286264731173, -294.4239320862337763, -309.3687407585708229 ) ) ;
#86101=CARTESIAN_POINT ( 'NONE',  ( 17.83663475847049185, -288.3442335507815528, -217.5776389324969387 ) ) ;
#86102=CARTESIAN_POINT ( 'NONE',  ( -115.3430155898818299, -287.8380690714489560, -288.1317622949166548 ) ) ;
#86103=CARTESIAN_POINT ( 'NONE',  ( -96.73340544276445030, -278.5579604239187574, -221.4945787034614568 ) ) ;
#86104=CARTESIAN_POINT ( 'NONE',  ( -103.3773380151498316, -286.0830144249798650, -305.6753559689226449 ) ) ;
#86105=CARTESIAN_POINT ( 'NONE',  ( -112.4158320185101019, -283.3096379623122516, -255.8565894072962124 ) ) ;
#86106=CARTESIAN_POINT ( 'NONE',  ( -66.92333195810844870, -287.5225718509133799, -338.7261009155925535 ) ) ;
#86107=CARTESIAN_POINT ( 'NONE',  ( 34.04525718381081134, -277.7398830232373257, -295.8971462202514999 ) ) ;
#86108=CARTESIAN_POINT ( 'NONE',  ( -38.08683333091465073, -274.3758427936994622, -197.3437757727656390 ) ) ;
#86110=CARTESIAN_POINT ( 'NONE',  ( -100.5828336845994926, -278.0509698189387677, -306.9257599442761943 ) ) ;
#86111=CARTESIAN_POINT ( 'NONE',  ( -43.75177264073350614, -279.3177332950034497, -197.4904620580578296 ) ) ;
#86112=CARTESIAN_POINT ( 'NONE',  ( 37.91276418562804196, -276.4463103103168464, -255.5875567493712879 ) ) ;
#86113=CARTESIAN_POINT ( 'NONE',  ( -88.65403744635321459, -278.1457016105900379, -213.4835938050755146 ) ) ;
#86114=CARTESIAN_POINT ( 'NONE',  ( -110.1644982457800950, -264.2653545926315815, -305.9146289097863587 ) ) ;
#86115=CARTESIAN_POINT ( 'NONE',  ( -34.12508696023863308, -275.0329281710281180, -193.6638324167203677 ) ) ;
#86116=CARTESIAN_POINT ( 'NONE',  ( -89.22166260746922717, -298.7647503922274836, -214.1906224796564686 ) ) ;
#86117=CARTESIAN_POINT ( 'NONE',  ( -85.33152481854864391, -287.9090924074130839, -210.2361428286349110 ) ) ;
#86119=CARTESIAN_POINT ( 'NONE',  ( 82.67040237643779221, -297.8655364536941192, -193.5104719492758534 ) ) ;
#86120=CARTESIAN_POINT ( 'NONE',  ( -37.29442038879642496, -287.1323945636266330, -197.0395286248191269 ) ) ;
#86121=CARTESIAN_POINT ( 'NONE',  ( -26.78436490224498456, -287.9446623775103831, -195.0586287482441037 ) ) ;
#86122=CARTESIAN_POINT ( 'NONE',  ( -8.185453708454760502, -288.0086602811940111, -337.4510853134514150 ) ) ;
#86123=CARTESIAN_POINT ( 'NONE',  ( -114.2791973961366381, -284.0646278548166492, -269.9758684761570180 ) ) ;
#86124=CARTESIAN_POINT ( 'NONE',  ( 15.84997504353883180, -279.2207327176601552, -219.1306275434438646 ) ) ;
#86125=CARTESIAN_POINT ( 'NONE',  ( 11.93659908474737641, -288.6056069137401323, -214.7716727209824796 ) ) ;
#86126=CARTESIAN_POINT ( 'NONE',  ( 36.11848389631552436, -280.1165700371992102, -276.8310959455851048 ) ) ;
#86127=CARTESIAN_POINT ( 'NONE',  ( -71.87116892264261026, -278.8337864708252027, -335.2518038767208282 ) ) ;
#86128=CARTESIAN_POINT ( 'NONE',  ( 25.32538962088364087, -275.5271033796352071, -232.7021973823910344 ) ) ;
#86129=CARTESIAN_POINT ( 'NONE',  ( -48.82470790767777657, -287.9900854451622081, -346.1521558340440379 ) ) ;
#86130=CARTESIAN_POINT ( 'NONE',  ( -95.20638058971513829, -284.6697830466758887, -320.9164102463781774 ) ) ;
#86131=CARTESIAN_POINT ( 'NONE',  ( -103.9902869537412187, -285.5457813836982837, -231.8169880328766794 ) ) ;
#86132=CARTESIAN_POINT ( 'NONE',  ( -32.96513488466632680, -280.2755050470740343, -197.4924300488215181 ) ) ;
#86136=CARTESIAN_POINT ( 'NONE',  ( -20.74355520701342215, -290.7018384893760867, -344.3392457607394022 ) ) ;
#86137=CARTESIAN_POINT ( 'NONE',  ( -109.4067231409171370, -288.9088678022301906, -296.2073931386224785 ) ) ;
#86138=CARTESIAN_POINT ( 'NONE',  ( -35.80106934112821904, -297.2690894033805193, -197.1998569180037180 ) ) ;
#86139=CARTESIAN_POINT ( 'NONE',  ( 38.50436707897962663, -293.0604840223909378, -283.1170848790582113 ) ) ;
#86140=CARTESIAN_POINT ( 'NONE',  ( -100.9117533263498672, -288.5238210972671595, -307.7384181341246858 ) ) ;
#86141=CARTESIAN_POINT ( 'NONE',  ( 15.61602450727186842, -291.0535285914015162, -218.5822398014605028 ) ) ;
#86142=CARTESIAN_POINT ( 'NONE',  ( 22.30534611916144172, -288.1616042857082221, -227.5044311724007002 ) ) ;
#86143=CARTESIAN_POINT ( 'NONE',  ( -106.6379572354042296, -298.6233781216988632, -303.7686719486574702 ) ) ;
#86144=CARTESIAN_POINT ( 'NONE',  ( 17.20810894700035476, -290.2739087980491490, -321.8326535991022297 ) ) ;
#86145=CARTESIAN_POINT ( 'NONE',  ( -112.5341989671727276, -288.5774064229840974, -268.3770677680075210 ) ) ;
#86146=CARTESIAN_POINT ( 'NONE',  ( 25.64437005843412010, -295.0025391302986577, -229.5513966709449676 ) ) ;
#86147=CARTESIAN_POINT ( 'NONE',  ( -66.64273944772145342, -284.3868933692981500, -337.4929671033554541 ) ) ;
#86148=CARTESIAN_POINT ( 'NONE',  ( -36.42689401635930579, -294.0637537354376718, -195.1872923611722399 ) ) ;
#86151=CARTESIAN_POINT ( 'NONE',  ( -93.86968991500313564, -275.2214292982374673, -220.5314764505885989 ) ) ;
#86152=CARTESIAN_POINT ( 'NONE',  ( -4.764424252452510444, -281.8088180449574338, -335.8693069671070361 ) ) ;
#86153=CARTESIAN_POINT ( 'NONE',  ( -56.86336323362571932, -281.3037452274124917, -342.7759321814564260 ) ) ;
#86154=CARTESIAN_POINT ( 'NONE',  ( -90.60752007190234281, -294.9807912191776609, -325.8140828105549076 ) ) ;
#86155=CARTESIAN_POINT ( 'NONE',  ( 33.84071785070673144, -273.5254679055530573, -249.9037296140886042 ) ) ;
#86156=CARTESIAN_POINT ( 'NONE',  ( -109.6834144956224435, -276.8590689206492925, -252.8114580486227680 ) ) ;
#86157=CARTESIAN_POINT ( 'NONE',  ( -40.55619145982202411, -299.3260977906836615, -196.9256643758872940 ) ) ;
#86158=CARTESIAN_POINT ( 'NONE',  ( -38.33216272160166938, -296.4900824633626826, -343.9436831916700044 ) ) ;
#86159=CARTESIAN_POINT ( 'NONE',  ( -58.44506725044026041, -296.1349072988235775, -340.4128818623713073 ) ) ;
#86162=CARTESIAN_POINT ( 'NONE',  ( 35.19415275998125026, -285.8342903664088794, -290.8279026627391204 ) ) ;
#86163=CARTESIAN_POINT ( 'NONE',  ( -103.2041632951744816, -272.8112449056056903, -238.8788062814458613 ) ) ;
#86164=CARTESIAN_POINT ( 'NONE',  ( -57.75593441690234187, -285.7957310267324260, -196.0611770603912873 ) ) ;
#86166=CARTESIAN_POINT ( 'NONE',  ( 35.92632655596987235, -287.5158921112999906, -293.9734147224672256 ) ) ;
#86167=CARTESIAN_POINT ( 'NONE',  ( 20.12990833785845979, -296.2033045184735442, -319.0994091516115532 ) ) ;
#86168=CARTESIAN_POINT ( 'NONE',  ( -16.90812760216920907, -290.3163318977087783, -198.3176333113612770 ) ) ;
#86169=CARTESIAN_POINT ( 'NONE',  ( -104.6472122639550975, -278.2304726642655055, -233.2919008856500511 ) ) ;
#86170=CARTESIAN_POINT ( 'NONE',  ( -106.6379572354042153, -294.4809262143061801, -236.9535640164627068 ) ) ;
#86172=CARTESIAN_POINT ( 'NONE',  ( -22.36389268175464906, -285.0430125300786699, -198.4563551109906427 ) ) ;
#86174=CARTESIAN_POINT ( 'NONE',  ( 17.45526775019607157, -286.2696054490617144, -321.6454079059366791 ) ) ;
#86175=CARTESIAN_POINT ( 'NONE',  ( -109.9252799767938882, -297.9772494752605212, -283.7750955080324502 ) ) ;
#86176=CARTESIAN_POINT ( 'NONE',  ( 19.67680657382954834, -282.2822394614445329, -219.4740122644367091 ) ) ;
#86177=CARTESIAN_POINT ( 'NONE',  ( -111.5155592359047176, -294.7421101762478770, -257.0703155336096870 ) ) ;
#86178=CARTESIAN_POINT ( 'NONE',  ( 15.82586250214500190, -282.2729679662205058, -320.4561446309208463 ) ) ;
#86179=CARTESIAN_POINT ( 'NONE',  ( -93.66420143866248793, -297.4352792401255101, -217.7783341986134360 ) ) ;
#86180=CARTESIAN_POINT ( 'NONE',  ( -58.11861974492182270, -299.2988921375849714, -199.6573177866117135 ) ) ;
#86181=CARTESIAN_POINT ( 'NONE',  ( -24.01538492022355342, -284.3007864750705949, -195.9323548680586384 ) ) ;
#86182=CARTESIAN_POINT ( 'NONE',  ( 22.96791733772884925, -282.9439607885518626, -225.7769201937584000 ) ) ;
#86184=CARTESIAN_POINT ( 'NONE',  ( -71.76503134961998853, -296.6442213188000210, -205.7060004631101435 ) ) ;
#86186=CARTESIAN_POINT ( 'NONE',  ( 10.99251291554320531, -284.3597662237326062, -327.3118916594960979 ) ) ;
#86188=CARTESIAN_POINT ( 'NONE',  ( -4.771743288812454686, -283.9809262143061233, -202.8022627189028810 ) ) ;
#86189=CARTESIAN_POINT ( 'NONE',  ( -9.280330824044447979, -275.8916553472793680, -341.8923585232664664 ) ) ;
#86190=CARTESIAN_POINT ( 'NONE',  ( 33.30873927388111611, -293.1429268588723858, -251.9895253233305255 ) ) ;
#86191=CARTESIAN_POINT ( 'NONE',  ( 36.39683177973545725, -283.0845964549790210, -271.3034874255757813 ) ) ;
#86192=CARTESIAN_POINT ( 'NONE',  ( 24.66752478077172839, -277.7013424890029683, -310.4715864164873551 ) ) ;
#86193=CARTESIAN_POINT ( 'NONE',  ( 24.47041098687520133, -283.7495474760008278, -314.9445061380191078 ) ) ;
#86194=CARTESIAN_POINT ( 'NONE',  ( 25.48407149801997917, -279.8263985856398222, -232.3145633146270086 ) ) ;
#86195=CARTESIAN_POINT ( 'NONE',  ( -86.39459255855943809, -279.7328562797914060, -327.1644876568187783 ) ) ;
#86196=CARTESIAN_POINT ( 'NONE',  ( -88.03796645749240213, -273.5327425011998912, -212.3343077688948597 ) ) ;
#86197=CARTESIAN_POINT ( 'NONE',  ( 39.13732681666608215, -275.5028936208451569, -279.7500034866696978 ) ) ;
#86198=CARTESIAN_POINT ( 'NONE',  ( 18.17042474618121872, -296.1681744956499642, -319.9758897439148768 ) ) ;
#86203=CARTESIAN_POINT ( 'NONE',  ( -6.325381000752239302, -292.7886205270276605, -339.4863191114410483 ) ) ;
#86204=CARTESIAN_POINT ( 'NONE',  ( -94.65708692226107246, -272.6986586816919385, -225.0517935722931497 ) ) ;
#86205=CARTESIAN_POINT ( 'NONE',  ( 37.67920192702032267, -295.2491966612953433, -284.3807215967667616 ) ) ;
#86206=CARTESIAN_POINT ( 'NONE',  ( -3.510615814643709864, -293.6938456423344519, -201.6191773866841572 ) ) ;
#86207=CARTESIAN_POINT ( 'NONE',  ( 11.32643419548897690, -290.3764556524163254, -327.2754204920393022 ) ) ;
#86208=CARTESIAN_POINT ( 'NONE',  ( -111.3079346288414797, -276.4058186468024587, -281.7200167399190036 ) ) ;
#86209=CARTESIAN_POINT ( 'NONE',  ( -37.79445049122723077, -278.9779828916521183, -344.8124441003350853 ) ) ;
#86210=CARTESIAN_POINT ( 'NONE',  ( 36.25802797991327253, -291.7806065219150469, -281.8489001126035305 ) ) ;
#86211=CARTESIAN_POINT ( 'NONE',  ( 22.75287375769195819, -282.7867761770912125, -224.1994110275627747 ) ) ;
#86212=CARTESIAN_POINT ( 'NONE',  ( -97.60222871350218554, -284.0519490281568551, -228.5909432129838592 ) ) ;
#86214=CARTESIAN_POINT ( 'NONE',  ( -6.027726585028406525, -282.2956631670616048, -336.3409431835260079 ) ) ;
#86215=CARTESIAN_POINT ( 'NONE',  ( -59.22713662753947972, -280.8549902806670957, -196.8592800582860605 ) ) ;
#86216=CARTESIAN_POINT ( 'NONE',  ( -111.9694047518493818, -283.5643574802977582, -253.0777611559296645 ) ) ;
#86217=CARTESIAN_POINT ( 'NONE',  ( -88.78268009777688974, -280.2916837429551720, -213.3817726710100260 ) ) ;
#86219=CARTESIAN_POINT ( 'NONE',  ( -110.0004737996372484, -279.7745651005986360, -293.8422694156296302 ) ) ;
#86221=CARTESIAN_POINT ( 'NONE',  ( 30.91033621190086578, -272.8380690714490129, -254.8156830097664738 ) ) ;
#86224=CARTESIAN_POINT ( 'NONE',  ( -44.79244279979960908, -299.9581344513669592, -195.6803591188261748 ) ) ;
#86225=CARTESIAN_POINT ( 'NONE',  ( -103.6046354759887294, -277.0306810199793404, -235.8819947378720769 ) ) ;
#86226=CARTESIAN_POINT ( 'NONE',  ( -113.1002435367726093, -292.2295619153871371, -276.8891450780491255 ) ) ;
#86227=CARTESIAN_POINT ( 'NONE',  ( 21.08025679689979626, -292.2845690747449225, -226.4206171030940595 ) ) ;
#86228=CARTESIAN_POINT ( 'NONE',  ( -85.13136277130155349, -289.1992434005931614, -330.7256556792448237 ) ) ;
#86229=CARTESIAN_POINT ( 'NONE',  ( 3.893926359213578881, -293.0836886467742488, -334.7524764141869582 ) ) ;
#86230=CARTESIAN_POINT ( 'NONE',  ( -81.94607671668215687, -283.8324531741836267, -211.5657950205414863 ) ) ;
#86231=CARTESIAN_POINT ( 'NONE',  ( 5.192298025046579113, -294.4942150562570191, -209.4563189778400840 ) ) ;
#86232=CARTESIAN_POINT ( 'NONE',  ( -70.42199879455813516, -284.8128070399175726, -336.0024501790110776 ) ) ;
#86233=CARTESIAN_POINT ( 'NONE',  ( -75.53617671055729943, -290.4900433667446578, -336.9494215471587495 ) ) ;
#86234=CARTESIAN_POINT ( 'NONE',  ( 13.37331014679241470, -281.2771943455525161, -217.6980724941505798 ) ) ;
#86235=CARTESIAN_POINT ( 'NONE',  ( -3.418501215188087361, -293.4092539862115814, -339.0577049524756603 ) ) ;
#86236=CARTESIAN_POINT ( 'NONE',  ( -28.98455913964636110, -289.7517491222019430, -346.7972331871446272 ) ) ;
#86237=CARTESIAN_POINT ( 'NONE',  ( -114.3284783354898480, -291.0335691076958256, -271.2343218690337494 ) ) ;
#86238=CARTESIAN_POINT ( 'NONE',  ( -94.12338067925827545, -285.3678566380152688, -224.4627619973549599 ) ) ;
#86241=CARTESIAN_POINT ( 'NONE',  ( 38.27119546791247018, -295.4832801221733121, -275.9244634561154612 ) ) ;
#86242=CARTESIAN_POINT ( 'NONE',  ( -95.21947267962707429, -294.5567454004556680, -320.3957231897343831 ) ) ;
#86243=CARTESIAN_POINT ( 'NONE',  ( -97.08456464264504859, -277.0210967274819041, -312.7408837310269405 ) ) ;
#86244=CARTESIAN_POINT ( 'NONE',  ( -112.3818752669307770, -272.2724018801275747, -253.3758591171066428 ) ) ;
#86245=CARTESIAN_POINT ( 'NONE',  ( -42.45699264858786393, -293.5977107771991541, -343.8767050057956567 ) ) ;
#86246=CARTESIAN_POINT ( 'NONE',  ( 19.76663549657548202, -276.6541510874912433, -223.2802087053597120 ) ) ;
#86247=CARTESIAN_POINT ( 'NONE',  ( -90.10370680157242873, -271.4361236336774255, -218.1400864786699572 ) ) ;
#86248=CARTESIAN_POINT ( 'NONE',  ( 33.50398087846112816, -295.0098380923572563, -289.5927894746005791 ) ) ;
#86249=CARTESIAN_POINT ( 'NONE',  ( -45.10987807316766407, -296.2323717831378076, -343.3081831533322656 ) ) ;
#86251=CARTESIAN_POINT ( 'NONE',  ( -111.3299248788238458, -294.7218451599225659, -257.1032513837006377 ) ) ;
#86252=CARTESIAN_POINT ( 'NONE',  ( -29.08157330243599148, -298.8044349271120836, -193.4621639557767878 ) ) ;
#86253=CARTESIAN_POINT ( 'NONE',  ( -5.554209228260244657, -287.2003123869359342, -336.7307672317078300 ) ) ;
#86255=CARTESIAN_POINT ( 'NONE',  ( -108.6593436259732073, -291.7130528629631385, -253.6570019851597806 ) ) ;
#86256=CARTESIAN_POINT ( 'NONE',  ( -76.40688607295069801, -274.0371025460335090, -204.0165398843044215 ) ) ;
#86257=CARTESIAN_POINT ( 'NONE',  ( -103.7395839019881834, -297.2965861191769932, -239.8517604270988954 ) ) ;
#86258=CARTESIAN_POINT ( 'NONE',  ( -112.7327660307813915, -280.5520720423783132, -268.7941583936683969 ) ) ;
#86259=CARTESIAN_POINT ( 'NONE',  ( 38.69462698084842600, -280.1244932509795262, -261.4243086426562286 ) ) ;
#86261=CARTESIAN_POINT ( 'NONE',  ( -44.41810874856214042, -282.4878974926833735, -346.9861833074120909 ) ) ;
#86262=CARTESIAN_POINT ( 'NONE',  ( 39.52918617465833506, -274.8751380959097901, -268.3167047885119132 ) ) ;
#86263=CARTESIAN_POINT ( 'NONE',  ( -28.29949838904284221, -278.5647978780119161, -194.6464405584155770 ) ) ;
#86264=CARTESIAN_POINT ( 'NONE',  ( 9.696073623395134788, -278.6971356703135712, -211.6643909721984471 ) ) ;
#86266=CARTESIAN_POINT ( 'NONE',  ( -47.32326030969229436, -296.6076257106947196, -197.4973938920623766 ) ) ;
#86267=CARTESIAN_POINT ( 'NONE',  ( -5.529903706810583408, -276.4707196843591532, -202.4280579822565187 ) ) ;
#86269=CARTESIAN_POINT ( 'NONE',  ( 21.83248970208357420, -290.9344367090293986, -223.6840633000784919 ) ) ;
#86270=CARTESIAN_POINT ( 'NONE',  ( -27.84909171997326638, -292.1693790550638141, -193.8948112050751149 ) ) ;
#86271=CARTESIAN_POINT ( 'NONE',  ( -8.562431834741454750, -278.6765642247831920, -339.8141182845718049 ) ) ;
#86272=CARTESIAN_POINT ( 'NONE',  ( -88.68438310270911984, -271.3319616250649347, -215.6189326606946111 ) ) ;
#86273=CARTESIAN_POINT ( 'NONE',  ( -102.3763532919609673, -284.2863313076109080, -229.4385971888172548 ) ) ;
#86275=CARTESIAN_POINT ( 'NONE',  ( -69.46683268374196984, -283.6292408607051811, -202.5756833079415458 ) ) ;
#86277=CARTESIAN_POINT ( 'NONE',  ( 35.59974763790477681, -292.4600517301558966, -278.9722793919557944 ) ) ;
#86278=CARTESIAN_POINT ( 'NONE',  ( -74.14780475061962761, -283.6971267830212469, -205.8779670114303997 ) ) ;
#86281=CARTESIAN_POINT ( 'NONE',  ( 18.55458807317983627, -292.2484930871154347, -320.3865286226737226 ) ) ;
#86282=CARTESIAN_POINT ( 'NONE',  ( -58.31493850242988941, -281.7981763255211831, -343.7838999290952984 ) ) ;
#86283=CARTESIAN_POINT ( 'NONE',  ( -24.75981994843965239, -281.8154854858634053, -197.6415421828658339 ) ) ;
#86284=CARTESIAN_POINT ( 'NONE',  ( -36.58484883322544334, -287.2665229466274468, -193.7489566462684536 ) ) ;
#86285=CARTESIAN_POINT ( 'NONE',  ( -5.349951678169219349, -278.7072058786992557, -201.4372320783726593 ) ) ;
#86286=CARTESIAN_POINT ( 'NONE',  ( 30.48518437149699878, -287.9149222174347074, -297.4884461264064157 ) ) ;
#86287=CARTESIAN_POINT ( 'NONE',  ( -29.63380325394025760, -278.3780643453470702, -343.5968823064588946 ) ) ;
#86288=CARTESIAN_POINT ( 'NONE',  ( -109.7831764641131684, -279.4943893598568820, -259.7703939831317825 ) ) ;
#86289=CARTESIAN_POINT ( 'NONE',  ( -24.10025114423919845, -288.2002050056193525, -196.1253768880712300 ) ) ;
#86291=CARTESIAN_POINT ( 'NONE',  ( -3.408379831611338062, -298.2993333195257151, -193.3620392314379899 ) ) ;
#86292=VECTOR ( 'NONE', #86880, 1000.000000000000000 ) ;
#86293=CARTESIAN_POINT ( 'NONE',  ( 17.23031493683589233, -290.2490159857565004, -321.3655699858621801 ) ) ;
#86295=CARTESIAN_POINT ( 'NONE',  ( -111.2869819898779866, -281.4805209788416960, -234.7871824221999191 ) ) ;
#86297=CARTESIAN_POINT ( 'NONE',  ( 6.194383980543309853, -272.6409561392168257, -209.0221268541379800 ) ) ;
#86298=CARTESIAN_POINT ( 'NONE',  ( 21.65418117016169575, -292.6064331404992913, -318.6094537536760072 ) ) ;
#86300=CARTESIAN_POINT ( 'NONE',  ( -38.65651086554108673, -287.5555284709033117, -196.6669122604396023 ) ) ;
#86301=CARTESIAN_POINT ( 'NONE',  ( 34.43284272088385478, -283.0765261195882090, -252.2434507622298270 ) ) ;
#86302=CARTESIAN_POINT ( 'NONE',  ( -97.68304183769218696, -291.3465170397900010, -317.2389248408354092 ) ) ;
#86303=CARTESIAN_POINT ( 'NONE',  ( 22.03309444367659253, -289.5189715471655632, -318.6303900393300523 ) ) ;
#86304=CARTESIAN_POINT ( 'NONE',  ( -110.6702582425654668, -286.3493563864115004, -286.1675975811750163 ) ) ;
#86305=CARTESIAN_POINT ( 'NONE',  ( -114.2109756558660507, -278.7749219013197717, -265.8762005561951582 ) ) ;
#86307=CARTESIAN_POINT ( 'NONE',  ( -55.74369649047332587, -293.3670965702268063, -343.6460463449091094 ) ) ;
#86308=CARTESIAN_POINT ( 'NONE',  ( 24.59300617215263784, -280.7774705281651109, -224.6107938304154175 ) ) ;
#86309=CARTESIAN_POINT ( 'NONE',  ( -101.8018897169095425, -274.9098867110279230, -233.4371889488425325 ) ) ;
#86310=CARTESIAN_POINT ( 'NONE',  ( -69.85430415644619018, -285.9805209788416391, -337.9475929042657754 ) ) ;
#86311=CARTESIAN_POINT ( 'NONE',  ( 24.51521640473169583, -273.1994078667647727, -226.2061425263158299 ) ) ;
#86313=CARTESIAN_POINT ( 'NONE',  ( -41.04804162620252583, -279.5119002925964082, -197.3936493785935511 ) ) ;
#86314=CARTESIAN_POINT ( 'NONE',  ( 37.82613986986537924, -276.5716943659761000, -255.6029151879837684 ) ) ;
#86315=CARTESIAN_POINT ( 'NONE',  ( -80.08491918998299752, -298.8860161893255167, -210.4579282516843364 ) ) ;
#86316=CARTESIAN_POINT ( 'NONE',  ( -69.10008882171740652, -282.5184739706987784, -340.2627195659547965 ) ) ;
#86317=CARTESIAN_POINT ( 'NONE',  ( -92.44234038387999419, -293.0099567477064966, -220.9266363056455305 ) ) ;
#86318=CARTESIAN_POINT ( 'NONE',  ( -34.15723516101967761, -275.6916980864387483, -194.2276851185533530 ) ) ;
#86319=CARTESIAN_POINT ( 'NONE',  ( 52.98980219858057694, -300.3645473847345784, -193.7401250667022907 ) ) ;
#86320=CARTESIAN_POINT ( 'NONE',  ( 36.65462921126223250, -295.7002883522731622, -281.8600899583505566 ) ) ;
#86321=CARTESIAN_POINT ( 'NONE',  ( -7.793200285562991603, -280.6638689061517198, -339.1136785590359182 ) ) ;
#86322=CARTESIAN_POINT ( 'NONE',  ( -110.4094861314438702, -290.5257626330152334, -245.9694937582152079 ) ) ;
#86323=CARTESIAN_POINT ( 'NONE',  ( 35.44309492666847916, -273.3579617242340305, -253.7442815901229665 ) ) ;
#86324=CARTESIAN_POINT ( 'NONE',  ( -7.673608376139617882, -288.0345627838862583, -200.1178468688961800 ) ) ;
#86326=CARTESIAN_POINT ( 'NONE',  ( -86.12451577205871445, -290.2773499221862608, -215.5711167681582197 ) ) ;
#86328=CARTESIAN_POINT ( 'NONE',  ( -111.3558588993663250, -288.8868463609599075, -289.4006274286459188 ) ) ;
#86329=CARTESIAN_POINT ( 'NONE',  ( -90.61108782081988977, -289.4996938909972641, -320.3795307763307960 ) ) ;
#86331=CARTESIAN_POINT ( 'NONE',  ( -43.65458900103428874, -287.0539592477167616, -193.8774504945046999 ) ) ;
#86332=CARTESIAN_POINT ( 'NONE',  ( -32.41489383520142553, -277.3217483603212941, -343.2658450267799140 ) ) ;
#86334=CARTESIAN_POINT ( 'NONE',  ( 37.15643751955254004, -292.7017875338705721, -288.6237164834165014 ) ) ;
#86335=CARTESIAN_POINT ( 'NONE',  ( -65.20750573733751310, -284.0583009951000690, -342.0468424071573850 ) ) ;
#86336=CARTESIAN_POINT ( 'NONE',  ( -112.1975920834811120, -284.6601343182347250, -288.3707270804216023 ) ) ;
#86337=CARTESIAN_POINT ( 'NONE',  ( -46.46330593507787654, -280.2666285908467785, -197.8608199629846069 ) ) ;
#86338=CARTESIAN_POINT ( 'NONE',  ( 168.1323214751145940, 232.5674794396639982, -192.7479069522925101 ) ) ;
#86339=CARTESIAN_POINT ( 'NONE',  ( -57.22704699613181845, -168.7833709488410818, -363.6107807818947890 ) ) ;
#86340=CARTESIAN_POINT ( 'NONE',  ( 195.2719850531713348, 282.9461876494999046, -110.4261502798884464 ) ) ;
#86342=CARTESIAN_POINT ( 'NONE',  ( -68.34171366185952934, -272.8314078624193826, -204.0782356775627875 ) ) ;
#86343=CARTESIAN_POINT ( 'NONE',  ( -8.838001346521661361, -273.3542176192941042, -202.7661315929888985 ) ) ;
#86344=CARTESIAN_POINT ( 'NONE',  ( -41.94814925529558280, -294.6162560650674322, -347.2139090605071488 ) ) ;
#86345=CARTESIAN_POINT ( 'NONE',  ( -106.9338212944154947, -265.3205186674255742, -305.6309630459658706 ) ) ;
#86346=CARTESIAN_POINT ( 'NONE',  ( -0.2696406066346856423, -273.2193269098884230, -203.4211815681448172 ) ) ;
#86347=CARTESIAN_POINT ( 'NONE',  ( -55.62034105952465524, -299.6749630383118301, -198.3582352620938707 ) ) ;
#86348=CARTESIAN_POINT ( 'NONE',  ( 28.67805875981774122, -289.3017653401319080, -302.6509757237433291 ) ) ;
#86349=CARTESIAN_POINT ( 'NONE',  ( -110.2818165302840043, -291.7283280005871120, -263.0149970709849754 ) ) ;
#86351=CARTESIAN_POINT ( 'NONE',  ( -114.0750813442570006, -297.5385987677553317, -266.7583135697273065 ) ) ;
#86352=CARTESIAN_POINT ( 'NONE',  ( -54.77709676717442022, -286.3144186711474504, -199.3581203944634126 ) ) ;
#86354=CARTESIAN_POINT ( 'NONE',  ( 13.29710821630033912, -295.1680795559121862, -328.2232806372514915 ) ) ;
#86355=CARTESIAN_POINT ( 'NONE',  ( 4.199353182774348880, -295.0009991585198463, -335.1839255148053098 ) ) ;
#86356=CARTESIAN_POINT ( 'NONE',  ( 2.238717458760330459, -292.7649171054112571, -208.9629101380651264 ) ) ;
#86358=CARTESIAN_POINT ( 'NONE',  ( -96.69736344339952439, -275.1095435563289584, -223.6040924685493678 ) ) ;
#86360=CARTESIAN_POINT ( 'NONE',  ( -112.0246671844481341, -278.2919511252330835, -251.8143463855297455 ) ) ;
#86361=CARTESIAN_POINT ( 'NONE',  ( -8.641102257194029690, -272.8338447037182277, -202.3160487866714448 ) ) ;
#86362=CARTESIAN_POINT ( 'NONE',  ( -36.49293769754876138, -299.2680872644565397, -196.9638634735345022 ) ) ;
#86363=CARTESIAN_POINT ( 'NONE',  ( 19.17280495417879038, -275.8353943621228268, -223.7830205100620162 ) ) ;
#86364=CARTESIAN_POINT ( 'NONE',  ( -63.23315966276098266, -275.4795684095734032, -198.9215887556935058 ) ) ;
#86366=CARTESIAN_POINT ( 'NONE',  ( 34.17707270369782435, -273.2650368110044496, -246.4589025258769936 ) ) ;
#86367=CARTESIAN_POINT ( 'NONE',  ( -67.32944891327855430, -296.1075192840649493, -337.0428826209879958 ) ) ;
#86368=CARTESIAN_POINT ( 'NONE',  ( 36.12415627872974966, -292.0605603591563977, -265.2937047847997292 ) ) ;
#86370=CARTESIAN_POINT ( 'NONE',  ( -103.3620152138814632, -279.5612256700283069, -230.7499842046176184 ) ) ;
#86371=CARTESIAN_POINT ( 'NONE',  ( -41.85446398826587711, -277.2772441112639399, -343.2340943474476376 ) ) ;
#86372=CARTESIAN_POINT ( 'NONE',  ( 39.08598663172784171, -286.1803768745480738, -265.8641857817764844 ) ) ;
#86373=CARTESIAN_POINT ( 'NONE',  ( -96.79982564474194362, -299.1813920034890657, -224.3538183514303626 ) ) ;
#86374=CARTESIAN_POINT ( 'NONE',  ( 82.67245219369620202, -297.7045441827060586, -197.0521791778547254 ) ) ;
#86375=CARTESIAN_POINT ( 'NONE',  ( 12.25778047535527371, -287.5379722566917167, -324.2118537354415366 ) ) ;
#86376=CARTESIAN_POINT ( 'NONE',  ( -110.6219054866518263, -276.9318290593772076, -259.6146442693682275 ) ) ;
#86377=CARTESIAN_POINT ( 'NONE',  ( -110.9398785623254895, -277.1594664548957780, -267.8703577606798376 ) ) ;
#86378=CARTESIAN_POINT ( 'NONE',  ( -47.52947603537365495, -285.1816843602759945, -344.7177447560963515 ) ) ;
#86379=CARTESIAN_POINT ( 'NONE',  ( 1.092359196607876948, -277.7321291609044351, -332.9504661303678859 ) ) ;
#86381=CARTESIAN_POINT ( 'NONE',  ( 36.51491496731624409, -273.7149207095698102, -251.6090294515939547 ) ) ;
#86382=CARTESIAN_POINT ( 'NONE',  ( 35.47896907995129823, -276.1119054076957013, -263.4028032306936211 ) ) ;
#86383=CARTESIAN_POINT ( 'NONE',  ( 35.88554643735736960, -283.3343134552551987, -253.3400180548439096 ) ) ;
#86385=CARTESIAN_POINT ( 'NONE',  ( 36.87117127708231124, -289.2912718827186040, -256.1567553334548393 ) ) ;
#86386=CARTESIAN_POINT ( 'NONE',  ( 37.60425367300548771, -291.6030440151465655, -274.3375138302612868 ) ) ;
#86388=CARTESIAN_POINT ( 'NONE',  ( -2.666285104127320338, -273.2056785842119098, -205.5625140479185973 ) ) ;
#86389=CARTESIAN_POINT ( 'NONE',  ( 36.43171639948916862, -291.8048171604463050, -279.0787236017769146 ) ) ;
#86390=CARTESIAN_POINT ( 'NONE',  ( -104.9628119525177112, -256.0684274861638983, -326.9234398911233939 ) ) ;
#86392=CARTESIAN_POINT ( 'NONE',  ( -111.5925778843774054, -288.8093070963093965, -288.0101205340813522 ) ) ;
#86393=CARTESIAN_POINT ( 'NONE',  ( -112.8986753436223154, -282.6897458480524961, -278.4306600278530937 ) ) ;
#86394=CARTESIAN_POINT ( 'NONE',  ( -29.36287170192303009, -284.3745221686216951, -343.5674341898863418 ) ) ;
#86395=CARTESIAN_POINT ( 'NONE',  ( -110.1561881557234415, -285.4552580112109581, -262.7433774483430966 ) ) ;
#86396=CARTESIAN_POINT ( 'NONE',  ( -85.48205720473674774, -293.3706654641899263, -212.3199657634946504 ) ) ;
#86397=CARTESIAN_POINT ( 'NONE',  ( -58.11999014631759053, -274.1242175615750511, -196.1841386552216022 ) ) ;
#86398=CARTESIAN_POINT ( 'NONE',  ( -92.55755105358264245, -287.9145728610459400, -322.0168201580793834 ) ) ;
#86399=CARTESIAN_POINT ( 'NONE',  ( -100.4655052535041477, -277.9692520710557915, -314.4563016933424819 ) ) ;
#86400=CARTESIAN_POINT ( 'NONE',  ( 34.89369184675017266, -295.2891519789712902, -251.5490220913792996 ) ) ;
#86402=CARTESIAN_POINT ( 'NONE',  ( -4.829096099716510437, -294.9805209788416391, -202.7746430608542312 ) ) ;
#86403=CARTESIAN_POINT ( 'NONE',  ( -98.50828509517155851, -283.7987756670174804, -229.6193413699363362 ) ) ;
#86404=CARTESIAN_POINT ( 'NONE',  ( -67.83541210034404401, -277.6518030914849078, -201.8260592758372525 ) ) ;
#86405=CARTESIAN_POINT ( 'NONE',  ( -9.454125105613082169, -296.7956549059167628, -194.1685552188437782 ) ) ;
#86406=CARTESIAN_POINT ( 'NONE',  ( 15.66608948680234548, -275.6253953390411766, -320.7006343524209910 ) ) ;
#86407=CARTESIAN_POINT ( 'NONE',  ( -37.57136222185162211, -293.5693853405915092, -196.6555783920228464 ) ) ;
#86408=CARTESIAN_POINT ( 'NONE',  ( 26.43357943670293153, -294.0009509561417644, -234.2559053233001691 ) ) ;
#86409=CARTESIAN_POINT ( 'NONE',  ( -94.27333152191833676, -297.1691917547461799, -321.4892180444213068 ) ) ;
#86410=CARTESIAN_POINT ( 'NONE',  ( -108.7786907208520546, -296.5844559066172224, -255.2758315196167018 ) ) ;
#86411=CARTESIAN_POINT ( 'NONE',  ( -81.56685075715807898, -291.6536940031137419, -330.9991267899555396 ) ) ;
#86412=CARTESIAN_POINT ( 'NONE',  ( -112.5246317212487099, -284.5108614525953499, -286.9902130148536799 ) ) ;
#86413=CARTESIAN_POINT ( 'NONE',  ( -60.47113307886002787, -271.8950508871518537, -198.1583805074809277 ) ) ;
#86414=CARTESIAN_POINT ( 'NONE',  ( 5.181444829031425670, -286.4430669223614814, -206.1042915139386196 ) ) ;
#86415=CARTESIAN_POINT ( 'NONE',  ( -106.7890561417611650, -280.1741229152506207, -297.7273662306832307 ) ) ;
#86416=CARTESIAN_POINT ( 'NONE',  ( -35.91690906059066890, -285.1292035160333853, -197.1396838308364750 ) ) ;
#86417=CARTESIAN_POINT ( 'NONE',  ( -90.20733976565934142, -287.7990660283465445, -323.6340576456236136 ) ) ;
#86418=CARTESIAN_POINT ( 'NONE',  ( 197.9738562182569694, 296.4636489450776367, -54.00000000000000711 ) ) ;
#86420=CARTESIAN_POINT ( 'NONE',  ( -101.0419038713099695, -284.5502215899518887, -234.4765566944677460 ) ) ;
#86422=CARTESIAN_POINT ( 'NONE',  ( 38.78635991060995281, -282.6443367673805369, -261.3811964523839606 ) ) ;
#86423=CARTESIAN_POINT ( 'NONE',  ( -48.84560911062249033, -288.2538667065797426, -346.3127265943128350 ) ) ;
#86424=CARTESIAN_POINT ( 'NONE',  ( -113.2799984448088395, -280.0648538424637763, -277.2789386874847537 ) ) ;
#86425=CARTESIAN_POINT ( 'NONE',  ( -81.96488948143928610, -280.7730444168118424, -208.2155691195069949 ) ) ;
#86426=CARTESIAN_POINT ( 'NONE',  ( -103.3689424359514248, -278.8075887693566415, -239.1070702138660522 ) ) ;
#86427=CARTESIAN_POINT ( 'NONE',  ( 24.81445327686541447, -292.9487465539360187, -224.9121070593207037 ) ) ;
#86428=CARTESIAN_POINT ( 'NONE',  ( -73.17000336490163193, -287.5497638199732364, -335.8453106671726687 ) ) ;
#86429=CARTESIAN_POINT ( 'NONE',  ( -39.21268854037838736, -293.6291943665424924, -194.1711890109491776 ) ) ;
#86430=CARTESIAN_POINT ( 'NONE',  ( -110.4085359659928400, -295.3864006520545900, -276.9136489945161657 ) ) ;
#86431=CARTESIAN_POINT ( 'NONE',  ( -26.50953543951491298, -284.8335650735134550, -344.0610956785242251 ) ) ;
#86432=CARTESIAN_POINT ( 'NONE',  ( -110.3953215218635791, -296.2404035640226425, -268.7281897585174306 ) ) ;
#86433=CARTESIAN_POINT ( 'NONE',  ( 38.05589761626159628, -294.8088172825385982, -284.4569336261859576 ) ) ;
#86434=CARTESIAN_POINT ( 'NONE',  ( 22.19169328058926283, -281.6117696140012185, -227.9386270418994513 ) ) ;
#86435=CARTESIAN_POINT ( 'NONE',  ( -13.12531760410572979, -273.4180151941861823, -197.5161659955479934 ) ) ;
#86436=CARTESIAN_POINT ( 'NONE',  ( -95.37591663605273595, -290.5207022480558976, -320.8125054870433814 ) ) ;
#86437=CARTESIAN_POINT ( 'NONE',  ( -4.717521196529470551, -280.7666336285604984, -338.7564252752937932 ) ) ;
#86438=CARTESIAN_POINT ( 'NONE',  ( -99.85061598318259257, -290.2895289752230497, -315.3100813557242077 ) ) ;
#86439=CARTESIAN_POINT ( 'NONE',  ( 15.98700896951612371, -287.1678475215834396, -220.4614456096433059 ) ) ;
#86441=CARTESIAN_POINT ( 'NONE',  ( -14.32388138225487850, -91.12230094864965224, -358.1431036431999360 ) ) ;
#86442=CARTESIAN_POINT ( 'NONE',  ( 184.1086675408331246, 260.7702122114448002, -150.9958300510270135 ) ) ;
#86443=CARTESIAN_POINT ( 'NONE',  ( -110.5535585741978508, -277.7457955153106468, -270.6284629835059263 ) ) ;
#86445=CARTESIAN_POINT ( 'NONE',  ( -99.72356926569732138, -278.0023733986776620, -231.7580913035668573 ) ) ;
#86446=CARTESIAN_POINT ( 'NONE',  ( -41.18746612208742874, -273.6718466802412308, -193.4261411279136382 ) ) ;
#86447=CARTESIAN_POINT ( 'NONE',  ( 140.3020133904481384, 178.1001207059538274, -239.2162932893931213 ) ) ;
#86448=CARTESIAN_POINT ( 'NONE',  ( -96.35072180182093859, -277.7842267615357628, -221.7965532727406242 ) ) ;
#86449=CARTESIAN_POINT ( 'NONE',  ( -36.19294861392245366, -281.0577873578358776, -344.9970823454893321 ) ) ;
#86450=CARTESIAN_POINT ( 'NONE',  ( -99.92891985083171846, -298.8889914382539246, -227.2474786046880695 ) ) ;
#86451=CARTESIAN_POINT ( 'NONE',  ( -96.81510487270033138, -291.6379222333050052, -227.8384916981444803 ) ) ;
#86452=CARTESIAN_POINT ( 'NONE',  ( -87.07534179161483223, -288.4467032014727010, -324.5393974894498115 ) ) ;
#86453=CARTESIAN_POINT ( 'NONE',  ( 18.01045344371307166, -275.4709783284677656, -216.9044312136182384 ) ) ;
#86454=CARTESIAN_POINT ( 'NONE',  ( -85.31016335348181201, -273.3677128144092876, -215.2662378431653565 ) ) ;
#86458=CARTESIAN_POINT ( 'NONE',  ( -74.32487172137903997, -281.4845176766745567, -204.4706086669636704 ) ) ;
#86460=CARTESIAN_POINT ( 'NONE',  ( -14.22438418033115859, -281.4386618551232004, -200.7386715428041271 ) ) ;
#86461=CARTESIAN_POINT ( 'NONE',  ( -74.53180612248333148, -281.3245306771157175, -204.0974776467722620 ) ) ;
#86462=CARTESIAN_POINT ( 'NONE',  ( -67.89341848551360670, -282.5220954481408739, -336.9193703201563608 ) ) ;
#86463=CARTESIAN_POINT ( 'NONE',  ( -106.4084820258049859, -280.0546659060465799, -297.5759138953037564 ) ) ;
#86464=CARTESIAN_POINT ( 'NONE',  ( -83.61101852201565521, -271.8837667750156015, -213.0038348717735914 ) ) ;
#86467=CARTESIAN_POINT ( 'NONE',  ( -74.01077179349272228, -278.3293864949231988, -337.9004387555592643 ) ) ;
#86469=CARTESIAN_POINT ( 'NONE',  ( -68.78958545139009573, -276.0322304367668949, -340.0147479401626356 ) ) ;
#86472=CARTESIAN_POINT ( 'NONE',  ( -109.5250025719447962, -286.2541195697757530, -292.0386652255925242 ) ) ;
#86473=CARTESIAN_POINT ( 'NONE',  ( 35.86951619082733345, -292.7547096577450816, -270.7710083561801753 ) ) ;
#86474=CARTESIAN_POINT ( 'NONE',  ( 30.26910897973711201, -287.3765443098334913, -307.1070236309670918 ) ) ;
#86475=CARTESIAN_POINT ( 'NONE',  ( -77.58145343362549795, -283.7442268206820017, -208.1815928474821078 ) ) ;
#86476=CARTESIAN_POINT ( 'NONE',  ( -52.19023546006646086, -284.4330281352165457, -198.2854916311188163 ) ) ;
#86477=CARTESIAN_POINT ( 'NONE',  ( 21.14459914411247965, -286.4223256483457476, -315.7393940265175161 ) ) ;
#86478=CARTESIAN_POINT ( 'NONE',  ( 36.10033822424737338, -282.7696009153808063, -271.3036252528334558 ) ) ;
#86479=CARTESIAN_POINT ( 'NONE',  ( -4.673614811919557965, -272.4822888465581059, -202.8355263023359214 ) ) ;
#86481=CARTESIAN_POINT ( 'NONE',  ( -70.69746270699212687, -284.0194350772653706, -201.8495604063347741 ) ) ;
#86482=CARTESIAN_POINT ( 'NONE',  ( -76.02818019034485530, -297.5686729813228339, -334.6738171867392566 ) ) ;
#86483=CARTESIAN_POINT ( 'NONE',  ( -15.91117444578450701, -284.3283997306367610, -198.2601021308670113 ) ) ;
#86485=CARTESIAN_POINT ( 'NONE',  ( -108.3974648963425409, -279.2595210641939047, -288.1465545297805306 ) ) ;
#86486=CARTESIAN_POINT ( 'NONE',  ( 27.11304886739153375, -289.0344757503367532, -231.5876226921864145 ) ) ;
#86491=CARTESIAN_POINT ( 'NONE',  ( 29.63739180786915384, -295.9320848867512268, -305.3341853160931691 ) ) ;
#86493=CARTESIAN_POINT ( 'NONE',  ( -112.1655873391877662, -276.4768869508372404, -276.2101703488430076 ) ) ;
#86494=CARTESIAN_POINT ( 'NONE',  ( -77.07698722531993951, -290.7315014170773679, -204.5330060143311641 ) ) ;
#86495=CARTESIAN_POINT ( 'NONE',  ( -45.19591361731023227, -293.5530039475170270, -343.7930159482908152 ) ) ;
#86496=CARTESIAN_POINT ( 'NONE',  ( -96.79485038647871420, -277.8375835803828977, -227.1573403322192632 ) ) ;
#86497=CARTESIAN_POINT ( 'NONE',  ( -84.07602035528144313, -271.4837990614615251, -212.4196172445070658 ) ) ;
#86498=CARTESIAN_POINT ( 'NONE',  ( -107.8732668597164519, -292.1392591447767586, -249.6635139811467354 ) ) ;
#86499=CARTESIAN_POINT ( 'NONE',  ( -106.6662871844225293, -281.4805209788416960, -237.0123917617630696 ) ) ;
#86500=CARTESIAN_POINT ( 'NONE',  ( -30.67101903103514360, -293.4491396299216603, -346.3756545275087433 ) ) ;
#86501=CARTESIAN_POINT ( 'NONE',  ( -2.975879951691980718, -290.1906082062209293, -335.7279916890816480 ) ) ;
#86502=CARTESIAN_POINT ( 'NONE',  ( 36.44342055898492561, -291.5618305230439091, -252.2026493786897561 ) ) ;
#86503=CARTESIAN_POINT ( 'NONE',  ( 24.01069576863294230, -289.5370241730160501, -311.0198220108498504 ) ) ;
#86505=CARTESIAN_POINT ( 'NONE',  ( -42.66548026638007940, -289.9237254767711534, -343.3793545533471843 ) ) ;
#86507=CARTESIAN_POINT ( 'NONE',  ( -38.89665040372960902, -290.2763240455488472, -346.9482634420761542 ) ) ;
#86508=CARTESIAN_POINT ( 'NONE',  ( 35.59334855745336768, -279.8145483121985535, -289.3053909708036713 ) ) ;
#86509=CARTESIAN_POINT ( 'NONE',  ( -107.7518858057029973, -290.8067722654363934, -251.0892277576016625 ) ) ;
#86510=CARTESIAN_POINT ( 'NONE',  ( -68.66780773178679453, -279.9848674493933345, -200.0301710753123245 ) ) ;
#86511=CARTESIAN_POINT ( 'NONE',  ( 33.54479863300238662, -281.6025070688658616, -300.5113676481673224 ) ) ;
#86512=CARTESIAN_POINT ( 'NONE',  ( 19.32022575039783874, -286.2343163765089002, -319.5756592770393922 ) ) ;
#86514=CARTESIAN_POINT ( 'NONE',  ( 35.91878273937629018, -279.8472731178611070, -282.3514111939365989 ) ) ;
#86515=CARTESIAN_POINT ( 'NONE',  ( -90.46785551010871984, -283.2996294836206630, -217.4214139592873209 ) ) ;
#86516=CARTESIAN_POINT ( 'NONE',  ( -106.7800878583809805, -277.4415715107390383, -238.5951022652082258 ) ) ;
#86517=CARTESIAN_POINT ( 'NONE',  ( -83.29993878155930531, -274.2063475022424086, -213.4362374268059455 ) ) ;
#86519=CARTESIAN_POINT ( 'NONE',  ( -111.1367662434341810, -292.1411499515317587, -271.2147162723267684 ) ) ;
#86520=CARTESIAN_POINT ( 'NONE',  ( 36.01501685001681352, -276.7050348262910688, -248.7894985191474859 ) ) ;
#86521=CARTESIAN_POINT ( 'NONE',  ( 26.78329200377127606, -275.6968005483327602, -305.3963521520410040 ) ) ;
#86522=CARTESIAN_POINT ( 'NONE',  ( -69.34833097464030516, -297.4733591768510905, -338.2027714645250853 ) ) ;
#86523=CARTESIAN_POINT ( 'NONE',  ( -74.42545568204182871, -289.6979756053364099, -337.8579842583397976 ) ) ;
#86524=CARTESIAN_POINT ( 'NONE',  ( 35.09112599277639077, -279.9091247010081815, -292.0536971579592205 ) ) ;
#86525=CARTESIAN_POINT ( 'NONE',  ( 28.05348044369287663, -292.8525756553774499, -229.6097766613948750 ) ) ;
#86526=CARTESIAN_POINT ( 'NONE',  ( -96.94589859175326296, -290.2045545953758392, -227.7224738577461096 ) ) ;
#86527=CARTESIAN_POINT ( 'NONE',  ( -58.31705146053971589, -293.3229525034639664, -342.4224412595595481 ) ) ;
#86530=CARTESIAN_POINT ( 'NONE',  ( -49.69296328023995812, -291.3981534834759941, -198.2997868370860033 ) ) ;
#86532=CARTESIAN_POINT ( 'NONE',  ( -21.39648532958014826, -280.3380690714490129, -340.3683826091709079 ) ) ;
#86533=CARTESIAN_POINT ( 'NONE',  ( -68.14280511368195903, -294.5056135763352358, -340.6754987677576310 ) ) ;
#86534=CARTESIAN_POINT ( 'NONE',  ( -68.96721297771652814, -284.7745350173466932, -340.0398135309175132 ) ) ;
#86535=CARTESIAN_POINT ( 'NONE',  ( -98.10589027291987918, -284.9470843605537880, -229.9048057365434659 ) ) ;
#86536=CARTESIAN_POINT ( 'NONE',  ( 27.38490336241590839, -277.5499053878468203, -305.6981520168409929 ) ) ;
#86537=CARTESIAN_POINT ( 'NONE',  ( 37.06195170961772334, -291.6496001805000446, -276.3563989471903710 ) ) ;
#86538=CARTESIAN_POINT ( 'NONE',  ( 35.90744663217885346, -295.1742726410018349, -259.7527951850630643 ) ) ;
#86539=CARTESIAN_POINT ( 'NONE',  ( -6.121590218001384365, -275.4274155596753531, -336.8011235376149557 ) ) ;
#86542=CARTESIAN_POINT ( 'NONE',  ( 22.26756620735826075, -293.8730753312837578, -319.0899163082253835 ) ) ;
#86543=CARTESIAN_POINT ( 'NONE',  ( 36.88987362935750269, -289.5527328293007372, -276.5777220055502426 ) ) ;
#86545=CARTESIAN_POINT ( 'NONE',  ( -99.25523899230893221, -274.3599914758804061, -225.1652414003027616 ) ) ;
#86546=CARTESIAN_POINT ( 'NONE',  ( -22.44716109393969816, -286.8992027657391191, -198.7406998100513533 ) ) ;
#86548=CARTESIAN_POINT ( 'NONE',  ( -74.88237176057604927, -278.6235736397393907, -203.4020395351702746 ) ) ;
#86549=CARTESIAN_POINT ( 'NONE',  ( 24.80879777540378228, -294.8056175612099423, -315.6671661990956750 ) ) ;
#86550=CARTESIAN_POINT ( 'NONE',  ( -15.33405060201770809, -286.9099416125969810, -342.9140302957284803 ) ) ;
#86551=CARTESIAN_POINT ( 'NONE',  ( -41.94005412120833398, -295.4417511395780025, -347.2548885691115856 ) ) ;
#86553=CARTESIAN_POINT ( 'NONE',  ( 16.75098663953888334, -293.1820872911092124, -221.2352683679915799 ) ) ;
#86558=CARTESIAN_POINT ( 'NONE',  ( -10.25831565879497198, -287.9192875929880415, -198.9662194095278664 ) ) ;
#86559=CARTESIAN_POINT ( 'NONE',  ( -72.02372285203398405, -283.1237833571631768, -198.2697987213421698 ) ) ;
#86561=AXIS2_PLACEMENT_3D ( 'NONE', #23037, #67078, #46204 ) ;
#86562=CARTESIAN_POINT ( 'NONE',  ( -98.49025049259559239, -278.5233984067970709, -223.7117009529606264 ) ) ;
#86563=CARTESIAN_POINT ( 'NONE',  ( -79.38615718651213626, -285.6214919280812978, -332.2666270668925108 ) ) ;
#86564=CARTESIAN_POINT ( 'NONE',  ( -65.64212688874044943, -284.2639610381068564, -199.3703719930022942 ) ) ;
#86566=CARTESIAN_POINT ( 'NONE',  ( 37.09489171929099172, -285.6412118374488500, -271.0738514758131714 ) ) ;
#86567=CARTESIAN_POINT ( 'NONE',  ( 30.75565881523614564, -277.8473004034264022, -303.6929674794075709 ) ) ;
#86568=CARTESIAN_POINT ( 'NONE',  ( -31.34220272111978289, -274.4632590561496386, -197.5742006228605874 ) ) ;
#86570=CARTESIAN_POINT ( 'NONE',  ( 32.81259321861030998, -292.5252439015642949, -292.2613144033559820 ) ) ;
#86571=CARTESIAN_POINT ( 'NONE',  ( -92.72663762731934867, -277.8750943379425280, -317.9164404838900282 ) ) ;
#86572=CARTESIAN_POINT ( 'NONE',  ( -66.10217463974014152, -279.0141250549779102, -203.1408555820492836 ) ) ;
#86573=CARTESIAN_POINT ( 'NONE',  ( 2.246617366452872577, -275.6490935848023014, -204.6781093158861040 ) ) ;
#86574=CARTESIAN_POINT ( 'NONE',  ( -112.6779380663107162, -277.1717738909307513, -284.3062580674422861 ) ) ;
#86575=CARTESIAN_POINT ( 'NONE',  ( 119.8472243494001503, 149.1509795950258876, -261.3511535428332877 ) ) ;
#86576=CARTESIAN_POINT ( 'NONE',  ( -71.79200863345266725, -296.9237957464192164, -338.5650954234693017 ) ) ;
#86578=CARTESIAN_POINT ( 'NONE',  ( 82.62999361571313273, -301.0392330995247789, -193.3423597593975956 ) ) ;
#86579=CARTESIAN_POINT ( 'NONE',  ( -104.8877006405983678, -286.0141680809398963, -241.7391104908703312 ) ) ;
#86580=CARTESIAN_POINT ( 'NONE',  ( -7.758601965761246610, -288.1945497742897828, -200.3136864427681019 ) ) ;
#86581=CARTESIAN_POINT ( 'NONE',  ( 19.58765224678785088, -287.5481978791106599, -316.2189581710816242 ) ) ;
#86582=CARTESIAN_POINT ( 'NONE',  ( -107.8672083172448311, -284.4536648349308052, -239.4760275200687829 ) ) ;
#86583=CARTESIAN_POINT ( 'NONE',  ( 13.90512840747237888, -279.1850558169803094, -217.1842997244860385 ) ) ;
#86584=CARTESIAN_POINT ( 'NONE',  ( -109.9228230600453600, -286.2096344421236154, -286.0049239099858482 ) ) ;
#86585=CARTESIAN_POINT ( 'NONE',  ( 19.38206654844255894, -279.3709616335137866, -223.2976951285214682 ) ) ;
#86586=CARTESIAN_POINT ( 'NONE',  ( -43.23001584571776590, -278.4432410717428752, -343.6180030938161849 ) ) ;
#86587=CARTESIAN_POINT ( 'NONE',  ( 33.56739263977607379, -275.8123980091436351, -252.7574534580762133 ) ) ;
#86588=CARTESIAN_POINT ( 'NONE',  ( -8.397461088183382216, -287.4764934968380317, -341.2994923637252214 ) ) ;
#86589=CARTESIAN_POINT ( 'NONE',  ( -55.65377196893206957, -284.0849025594745285, -344.9856906439463273 ) ) ;
#86590=CIRCLE ( 'NONE', #12537, 6.154241149514405151 ) ;
#86591=CARTESIAN_POINT ( 'NONE',  ( 32.33932048692548733, -282.4639266343517647, -303.1069315509960234 ) ) ;
#86595=CARTESIAN_POINT ( 'NONE',  ( -67.53944006126283739, -291.3045185465318241, -339.8478216424853144 ) ) ;
#86596=CARTESIAN_POINT ( 'NONE',  ( -113.1750209137404397, -289.3693546684516491, -259.8444448273807552 ) ) ;
#86597=CARTESIAN_POINT ( 'NONE',  ( -98.03147786611464198, -272.1798973711223653, -229.2809214978196053 ) ) ;
#86599=CARTESIAN_POINT ( 'NONE',  ( 36.99589893742542301, -293.1474253915205850, -290.0393839646713445 ) ) ;
#86600=CARTESIAN_POINT ( 'NONE',  ( -111.0608795363489776, -289.0573305001290692, -268.4244046645557091 ) ) ;
#86601=CARTESIAN_POINT ( 'NONE',  ( 19.26589789839507461, -291.1238969545192958, -222.6793199731177140 ) ) ;
#86602=CARTESIAN_POINT ( 'NONE',  ( 16.31165787213243235, -289.4743245370594309, -320.5199069232691613 ) ) ;
#86603=CARTESIAN_POINT ( 'NONE',  ( -69.85430415644619018, -297.9805209788416391, -337.9475929042657754 ) ) ;
#86604=CARTESIAN_POINT ( 'NONE',  ( 22.56059550323598373, -290.1692442202887605, -315.4911039126819219 ) ) ;
#86605=CARTESIAN_POINT ( 'NONE',  ( -112.2867767625877207, -288.4698658295511677, -276.7712763467328045 ) ) ;
#86606=CARTESIAN_POINT ( 'NONE',  ( -71.84811252851179120, -293.5962634241609521, -203.7563775444847352 ) ) ;
#86607=CARTESIAN_POINT ( 'NONE',  ( -103.2190963056276729, -285.0602782140209683, -302.4709360955877742 ) ) ;
#86608=CARTESIAN_POINT ( 'NONE',  ( 37.82176059342154417, -295.5154156594693973, -267.4808256001151108 ) ) ;
#86609=CARTESIAN_POINT ( 'NONE',  ( -114.0438498160389287, -273.6021560138187851, -270.3744733279939965 ) ) ;
#86612=CARTESIAN_POINT ( 'NONE',  ( -104.1623545849157608, -274.9924854991103871, -235.4142766501725816 ) ) ;
#86613=CARTESIAN_POINT ( 'NONE',  ( 34.72791690778539930, -280.5835666836326823, -257.7685794157575856 ) ) ;
#86614=CARTESIAN_POINT ( 'NONE',  ( -88.30606934901378224, -281.7653921865735924, -325.4561296543740241 ) ) ;
#86615=CARTESIAN_POINT ( 'NONE',  ( -109.6953663863599360, -296.0765333812132099, -244.4940385337762905 ) ) ;
#86616=CARTESIAN_POINT ( 'NONE',  ( -36.70514686350039568, -272.3001141793175748, -196.3379308233194251 ) ) ;
#86617=CARTESIAN_POINT ( 'NONE',  ( -103.1409666945161376, -276.1670178666419702, -305.1716151698924477 ) ) ;
#86618=CARTESIAN_POINT ( 'NONE',  ( -44.63457604021047587, -299.2732584249731076, -197.1799815692015443 ) ) ;
#86620=CARTESIAN_POINT ( 'NONE',  ( -23.38947313059208710, -296.2956951785070032, -342.6676235240379924 ) ) ;
#86621=CARTESIAN_POINT ( 'NONE',  ( -70.99599795410820491, -296.3109421953061542, -335.3365823052049564 ) ) ;
#86624=CARTESIAN_POINT ( 'NONE',  ( 37.95935206350324620, -285.6233772988311443, -274.3613093923165138 ) ) ;
#86625=CARTESIAN_POINT ( 'NONE',  ( -109.0456709670273057, -296.7336842046639163, -256.5999975610927208 ) ) ;
#86626=VECTOR ( 'NONE', #90075, 1000.000000000000000 ) ;
#86627=CARTESIAN_POINT ( 'NONE',  ( -100.9964917951645447, -285.1245554816696881, -226.9417931976975638 ) ) ;
#86628=CARTESIAN_POINT ( 'NONE',  ( 38.27021368908083332, -287.0382009155877086, -255.9187227345602764 ) ) ;
#86629=CARTESIAN_POINT ( 'NONE',  ( -89.55385694715241129, -297.7630677471756826, -324.7679817973432250 ) ) ;
#86630=CARTESIAN_POINT ( 'NONE',  ( 31.55332648678318108, -291.1678279917462078, -241.0136516255639663 ) ) ;
#86632=CARTESIAN_POINT ( 'NONE',  ( -25.41056192972533623, -279.3977002205458575, -194.4545519860903937 ) ) ;
#86633=CARTESIAN_POINT ( 'NONE',  ( 21.27581636871891391, -279.6952119285918457, -317.1477375740089997 ) ) ;
#86636=CARTESIAN_POINT ( 'NONE',  ( -6.837553730355165449, -285.2566054092299055, -203.5893374466559465 ) ) ;
#86637=CARTESIAN_POINT ( 'NONE',  ( -87.19397867757579945, -288.6479529970536078, -328.7081736748474441 ) ) ;
#86639=CARTESIAN_POINT ( 'NONE',  ( 129.8483263487583201, -299.5541904835127980, -195.3611179825600175 ) ) ;
#86640=CARTESIAN_POINT ( 'NONE',  ( -105.6952829210544991, -297.7835847718082505, -298.1860731998385745 ) ) ;
#86641=CARTESIAN_POINT ( 'NONE',  ( -72.25390656051285987, -281.0247557833624796, -202.3778776701827269 ) ) ;
#86642=CARTESIAN_POINT ( 'NONE',  ( -107.9063864159121806, -294.2288382810562553, -296.9476805277259928 ) ) ;
#86643=CARTESIAN_POINT ( 'NONE',  ( 22.13317929003263984, -280.6272342822693986, -227.9957287477335512 ) ) ;
#86644=CARTESIAN_POINT ( 'NONE',  ( -0.7043056518484719364, -294.7459482385098113, -338.1011932398528756 ) ) ;
#86646=CARTESIAN_POINT ( 'NONE',  ( -110.8287231321905040, -280.3590449753974099, -285.4130816221634177 ) ) ;
#86647=CARTESIAN_POINT ( 'NONE',  ( -79.85492834090354108, -296.5198728734865199, -210.7286278917784728 ) ) ;
#86651=CARTESIAN_POINT ( 'NONE',  ( -0.4169210472922616484, -284.5385596007845947, -335.2333577570809666 ) ) ;
#86653=CARTESIAN_POINT ( 'NONE',  ( -106.6662871844225293, -287.6237833571633473, -303.7098442033569086 ) ) ;
#86654=CARTESIAN_POINT ( 'NONE',  ( -7.955868606643791807, -275.8740238432718570, -341.3727782244550895 ) ) ;
#86655=CARTESIAN_POINT ( 'NONE',  ( 16.73960894791003184, -292.6822067836282031, -221.2542117713003620 ) ) ;
#86656=CARTESIAN_POINT ( 'NONE',  ( 33.39472534701439344, -282.8014630031112233, -249.6955460279457384 ) ) ;
#86657=CARTESIAN_POINT ( 'NONE',  ( -38.11092209400543851, -275.6424849317033932, -196.5651240865178409 ) ) ;
#86659=CARTESIAN_POINT ( 'NONE',  ( 4.127594721337612960, -284.1038895794540053, -334.3510906276478067 ) ) ;
#86660=CARTESIAN_POINT ( 'NONE',  ( 21.65725855215440987, -279.7380021454428061, -226.6792975752978521 ) ) ;
#86661=CARTESIAN_POINT ( 'NONE',  ( -107.1194733263091479, -280.1943879412970659, -297.8577180270788745 ) ) ;
#86662=CARTESIAN_POINT ( 'NONE',  ( -81.25212869392009907, -273.6403449735436766, -207.0440409089503078 ) ) ;
#86663=CARTESIAN_POINT ( 'NONE',  ( 29.94856527696839876, -274.8990454977193281, -232.8212673127507912 ) ) ;
#86664=CARTESIAN_POINT ( 'NONE',  ( 19.07955243041028126, -296.1506179762771467, -318.9393553440310143 ) ) ;
#86667=CARTESIAN_POINT ( 'NONE',  ( 10.40128966923078302, -292.5411853387999486, -329.2582298398679086 ) ) ;
#86668=CARTESIAN_POINT ( 'NONE',  ( -71.93133220182700427, -273.0898281975242412, -205.9499056625479341 ) ) ;
#86669=CARTESIAN_POINT ( 'NONE',  ( 22.55171687390224022, -294.4338839230368876, -223.0593153689044073 ) ) ;
#86670=CARTESIAN_POINT ( 'NONE',  ( -99.90806341382572953, -299.6948066931273047, -220.5068182859052968 ) ) ;
#86671=CARTESIAN_POINT ( 'NONE',  ( -34.98806743517886275, -293.2861335694759077, -193.7812730045262981 ) ) ;
#86672=CARTESIAN_POINT ( 'NONE',  ( 20.95738955222951105, -290.1993422388954400, -317.2785409040520790 ) ) ;
#86673=CARTESIAN_POINT ( 'NONE',  ( -109.5969203092538322, -276.3010762879391677, -289.8344737676102341 ) ) ;
#86674=CARTESIAN_POINT ( 'NONE',  ( -56.95651819445507869, -279.2271161602518532, -342.2239288787270652 ) ) ;
#86675=CARTESIAN_POINT ( 'NONE',  ( 36.13926416016368393, -291.4768814131369368, -258.3706629114885800 ) ) ;
#86676=CARTESIAN_POINT ( 'NONE',  ( 3.141622936810263500, -282.4497111881916567, -206.2569376537458936 ) ) ;
#86678=CARTESIAN_POINT ( 'NONE',  ( 5.601101455435562926, -282.1188570139379976, -329.4204379824330431 ) ) ;
#86679=CARTESIAN_POINT ( 'NONE',  ( -41.00743043545369915, -281.0867354221526284, -193.7447449540067339 ) ) ;
#86681=CARTESIAN_POINT ( 'NONE',  ( -95.97633632999615827, -282.6796996051750739, -319.6763288866721382 ) ) ;
#86682=CARTESIAN_POINT ( 'NONE',  ( -97.51993451947126346, -280.1330867536838127, -222.7019077526034323 ) ) ;
#86684=CARTESIAN_POINT ( 'NONE',  ( 38.23478642177757791, -276.9393692068623523, -259.8300955601204123 ) ) ;
#86685=CARTESIAN_POINT ( 'NONE',  ( -92.05005921254146983, -286.4090924074130839, -314.0302885647153062 ) ) ;
#86689=CARTESIAN_POINT ( 'NONE',  ( -66.36968767766522603, -299.6722401657189039, -201.2063886482227701 ) ) ;
#86691=CARTESIAN_POINT ( 'NONE',  ( -59.71140343208254819, -275.3634594636380371, -341.5751838313061626 ) ) ;
#86692=CARTESIAN_POINT ( 'NONE',  ( -110.6610301073443736, -292.5661275606721574, -250.3554912141422903 ) ) ;
#86693=CARTESIAN_POINT ( 'NONE',  ( 34.81589721817466199, -292.7454174113557883, -258.5706659591877496 ) ) ;
#86694=CARTESIAN_POINT ( 'NONE',  ( -112.5065677701033167, -289.8542303650173722, -286.7857816292012103 ) ) ;
#86696=CARTESIAN_POINT ( 'NONE',  ( -53.18493490559410475, -293.8260492327401607, -345.1654854126097121 ) ) ;
#86697=CARTESIAN_POINT ( 'NONE',  ( -98.76169625675011332, -283.5138672670969413, -229.4462736011043944 ) ) ;
#86698=CARTESIAN_POINT ( 'NONE',  ( -97.78057896873443156, -293.0057700165469328, -227.1695229211751439 ) ) ;
#86699=CARTESIAN_POINT ( 'NONE',  ( -9.210978061590564536, -284.9065961328348635, -202.2345573385242119 ) ) ;
#86700=CARTESIAN_POINT ( 'NONE',  ( 1.375247953333307738, -283.8386693197529098, -332.8884730680869666 ) ) ;
#86701=CARTESIAN_POINT ( 'NONE',  ( -112.8995707007084945, -291.3223842879201015, -283.9936348109647497 ) ) ;
#86702=CARTESIAN_POINT ( 'NONE',  ( 34.62662783376197240, -281.8785372207613023, -257.7695250671700364 ) ) ;
#86703=CARTESIAN_POINT ( 'NONE',  ( -0.9086171950829795563, -293.3744140845097377, -337.7601903255441584 ) ) ;
#86704=CARTESIAN_POINT ( 'NONE',  ( 5.475836976171089887, -289.2911366344806083, -334.1640750962648099 ) ) ;
#86705=CARTESIAN_POINT ( 'NONE',  ( 23.24288397586526500, -288.6790875584675291, -317.8063261126611110 ) ) ;
#86706=CARTESIAN_POINT ( 'NONE',  ( -69.98433501684097280, -285.7764693340060376, -205.0520100612092733 ) ) ;
#86708=DIRECTION ( 'NONE',  ( 1.000000000000000000, 0.000000000000000000, 0.000000000000000000 ) ) ;
#86709=CARTESIAN_POINT ( 'NONE',  ( -3.754695127627726059, -296.4742495132108502, -338.2888061178431371 ) ) ;
#86711=CARTESIAN_POINT ( 'NONE',  ( -108.9817021583558017, -294.8934493970625681, -297.3622740399097779 ) ) ;
#86712=CARTESIAN_POINT ( 'NONE',  ( -110.6274337749806733, -277.6073983759084740, -270.6269837945009158 ) ) ;
#86714=CARTESIAN_POINT ( 'NONE',  ( -114.1191532768571619, -272.1316067803842316, -264.6245811096715101 ) ) ;
#86715=CARTESIAN_POINT ( 'NONE',  ( -15.40472209019244154, -293.2429894010492717, -340.7673072040351485 ) ) ;
#86716=CARTESIAN_POINT ( 'NONE',  ( 3.470279454689859655, -276.3689327198972592, -208.5555960561645463 ) ) ;
#86717=CARTESIAN_POINT ( 'NONE',  ( -57.16910997214898060, -271.9333435231922067, -198.7691379592928627 ) ) ;
#86718=CARTESIAN_POINT ( 'NONE',  ( 27.83212250028824997, -294.3006420160401149, -236.6045875376940444 ) ) ;
#86719=CARTESIAN_POINT ( 'NONE',  ( -88.70867372903639136, -296.8732738897116974, -322.7359824693222663 ) ) ;
#86722=CARTESIAN_POINT ( 'NONE',  ( -112.4759463231367675, -294.5976597225312048, -266.7962079353489457 ) ) ;
#86723=CARTESIAN_POINT ( 'NONE',  ( -34.06070296774593942, -298.7436293451507368, -193.4626981786925342 ) ) ;
#86724=CARTESIAN_POINT ( 'NONE',  ( -111.1012288709428191, -274.7303055157603353, -256.4985364200303479 ) ) ;
#86725=CARTESIAN_POINT ( 'NONE',  ( -98.29989936894735081, -290.9314815426498626, -310.9734290032396302 ) ) ;
#86726=CARTESIAN_POINT ( 'NONE',  ( 3.831806899958924539, -294.8139180827574251, -330.6672520463549176 ) ) ;
#86727=CARTESIAN_POINT ( 'NONE',  ( -111.4434848272890264, -280.3562271081813151, -284.1188251430195919 ) ) ;
#86728=CARTESIAN_POINT ( 'NONE',  ( -64.55117762688779237, -278.3892292071748784, -198.8004110773277091 ) ) ;
#86730=CARTESIAN_POINT ( 'NONE',  ( -63.88462517043102906, -282.7379730644068445, -342.5330371526828230 ) ) ;
#86731=CARTESIAN_POINT ( 'NONE',  ( 14.80795133416751952, -275.6891104146346834, -326.9466496730910876 ) ) ;
#86732=CARTESIAN_POINT ( 'NONE',  ( -107.7654563252636848, -277.3258044046063446, -241.2589706949641197 ) ) ;
#86733=CARTESIAN_POINT ( 'NONE',  ( -31.19759255770202699, -278.1293027332055203, -195.3945408290494754 ) ) ;
#86734=ADVANCED_FACE ( 'NONE', ( #67248, #52544 ), #89441, .T. ) ;
#86735=CARTESIAN_POINT ( 'NONE',  ( -50.02265937824991937, -296.5717627639884313, -197.9702570311816032 ) ) ;
#86736=CARTESIAN_POINT ( 'NONE',  ( 37.70677765558541950, -277.5439293079206209, -269.7078477727451400 ) ) ;
#86738=CARTESIAN_POINT ( 'NONE',  ( -66.35828801208229777, -289.6942219311950453, -200.8165680025540496 ) ) ;
#86739=CARTESIAN_POINT ( 'NONE',  ( -112.3172705891065988, -290.7715247174101023, -252.8207692390531065 ) ) ;
#86740=CARTESIAN_POINT ( 'NONE',  ( -75.52394515027168609, -275.5446726040855197, -205.5541919999960783 ) ) ;
#86741=CARTESIAN_POINT ( 'NONE',  ( -71.27671329616893559, -295.6029625535011860, -203.6502075215037735 ) ) ;
#86742=CARTESIAN_POINT ( 'NONE',  ( -40.79895115453716414, -285.2070089660477379, -193.5483263464104482 ) ) ;
#86744=CARTESIAN_POINT ( 'NONE',  ( -99.86092609266262343, -281.9913932701669523, -311.8814526483932354 ) ) ;
#86746=CARTESIAN_POINT ( 'NONE',  ( 6.927883640651658403, -291.4651308904388998, -211.8176772176007887 ) ) ;
#86747=CARTESIAN_POINT ( 'NONE',  ( -94.18591574876103323, -283.3585247542855541, -222.6159545265933843 ) ) ;
#86750=CARTESIAN_POINT ( 'NONE',  ( 3.346337345427247367, -290.5984256856759202, -207.2957419298513173 ) ) ;
#86751=CARTESIAN_POINT ( 'NONE',  ( -110.4493271790812088, -282.7546704188016520, -292.2693443716538582 ) ) ;
#86752=CARTESIAN_POINT ( 'NONE',  ( -21.46122829231144635, -278.4453977070242559, -342.4848360931924276 ) ) ;
#86753=CARTESIAN_POINT ( 'NONE',  ( -43.64895670453570631, -287.1793433499586854, -193.9653060778406370 ) ) ;
#86754=CARTESIAN_POINT ( 'NONE',  ( 33.08190655882897602, -287.8083413300794859, -289.7714889439299100 ) ) ;
#86755=CARTESIAN_POINT ( 'NONE',  ( -56.73814154964617984, -278.7323140456948636, -341.4010271746753347 ) ) ;
#86756=CARTESIAN_POINT ( 'NONE',  ( -97.01148390475290739, -278.7648996115511864, -312.7162937232749300 ) ) ;
#86757=CARTESIAN_POINT ( 'NONE',  ( -77.47433449402109318, -287.5138048364202632, -207.0020436016884844 ) ) ;
#86760=CARTESIAN_POINT ( 'NONE',  ( -110.8124856383814034, -296.6770208126011426, -247.1400003917706272 ) ) ;
#86761=CARTESIAN_POINT ( 'NONE',  ( -0.1505256645194337772, -290.5351261920225738, -335.1405081192834245 ) ) ;
#86763=CARTESIAN_POINT ( 'NONE',  ( -111.2869819898779866, -287.4805209788416391, -234.7871824221999191 ) ) ;
#86765=CARTESIAN_POINT ( 'NONE',  ( 38.06331026441004894, -291.8088035336748476, -259.0280594007051604 ) ) ;
#86767=CARTESIAN_POINT ( 'NONE',  ( 19.18121083802451565, -288.4071935035355523, -223.0564963105121592 ) ) ;
#86769=CARTESIAN_POINT ( 'NONE',  ( 32.01209631713407333, -282.9705450988461166, -244.3680249718194943 ) ) ;
#86770=CARTESIAN_POINT ( 'NONE',  ( 18.22885088892227046, -289.6991133662497191, -322.8065196151509895 ) ) ;
#86771=CARTESIAN_POINT ( 'NONE',  ( 36.31421764920121831, -289.1288242860660489, -291.0998763137836818 ) ) ;
#86772=CARTESIAN_POINT ( 'NONE',  ( -110.3669567502479509, -286.3321290563596904, -287.5142968913292520 ) ) ;
#86773=CARTESIAN_POINT ( 'NONE',  ( -95.20938898244470749, -278.0314176480131323, -321.1580725288027907 ) ) ;
#86775=CARTESIAN_POINT ( 'NONE',  ( -27.95149810235949772, -293.0138097048730970, -345.3876637607737621 ) ) ;
#86776=CARTESIAN_POINT ( 'NONE',  ( 28.30389320523857322, -281.9124432975543755, -310.7071090440763328 ) ) ;
#86778=CARTESIAN_POINT ( 'NONE',  ( -98.88019599209147259, -274.9811132730073382, -228.7497480662936766 ) ) ;
#86781=CARTESIAN_POINT ( 'NONE',  ( 31.95455697924148097, -289.6233781216988064, -236.9535640164627637 ) ) ;
#86782=CARTESIAN_POINT ( 'NONE',  ( -64.51647401274645688, -271.9421256445228323, -199.3858237804838609 ) ) ;
#86784=CARTESIAN_POINT ( 'NONE',  ( -100.8622202828733663, -278.5537948022475803, -234.2621988743837278 ) ) ;
#86785=CARTESIAN_POINT ( 'NONE',  ( 36.20029734389860465, -276.4848738137167743, -248.7379886606918262 ) ) ;
#86786=CARTESIAN_POINT ( 'NONE',  ( -60.72015274471441160, -299.1682260567342269, -200.5302615611704766 ) ) ;
#86787=CARTESIAN_POINT ( 'NONE',  ( -109.0873391921046078, -283.2625887709342010, -297.8110137020640877 ) ) ;
#86788=CARTESIAN_POINT ( 'NONE',  ( -102.5251139082621847, -291.8394605150623420, -305.5281926994011314 ) ) ;
#86789=CARTESIAN_POINT ( 'NONE',  ( 30.00702508275892200, -300.4010117140515490, -194.0373803870615461 ) ) ;
#86790=CARTESIAN_POINT ( 'NONE',  ( -23.46477283104988132, -299.4273271954446045, -193.7554179349797892 ) ) ;
#86791=CARTESIAN_POINT ( 'NONE',  ( 27.39099520683090461, -296.0547708562792195, -307.9071774166563955 ) ) ;
#86792=CARTESIAN_POINT ( 'NONE',  ( -110.2163411749519497, -282.3324557182195917, -287.4264551373652239 ) ) ;
#86793=CARTESIAN_POINT ( 'NONE',  ( -105.9833334332431605, -290.6689138343548393, -235.4000849822964199 ) ) ;
#86794=CARTESIAN_POINT ( 'NONE',  ( -66.43140005271798998, -271.6894408729166912, -201.6178553100715192 ) ) ;
#86795=CARTESIAN_POINT ( 'NONE',  ( -52.03915023367822812, -287.4673228406683165, -195.5381428955062404 ) ) ;
#86797=CARTESIAN_POINT ( 'NONE',  ( -109.7265047859118994, -289.3190001243189045, -282.0447395844415155 ) ) ;
#86798=CARTESIAN_POINT ( 'NONE',  ( 26.75917060119040514, -23.72314211615959323, -344.9376292452095640 ) ) ;
#86800=CARTESIAN_POINT ( 'NONE',  ( -95.20276076680376320, -289.8062189588819137, -220.4341717469561956 ) ) ;
#86801=CARTESIAN_POINT ( 'NONE',  ( 24.25390665540478707, -287.7609755527370794, -309.5793371125305384 ) ) ;
#86803=CARTESIAN_POINT ( 'NONE',  ( -30.92348114642763690, -287.2111067028664593, -193.9260277965745729 ) ) ;
#86804=CARTESIAN_POINT ( 'NONE',  ( -5.052915407156727490, -276.9482994221830836, -335.8694542499625868 ) ) ;
#86805=EDGE_CURVE ( 'NONE', #19844, #8997, #3740, .T. ) ;
#86806=CARTESIAN_POINT ( 'NONE',  ( 39.34742160862095517, -292.4360794352614334, -267.4620593073188388 ) ) ;
#86807=CARTESIAN_POINT ( 'NONE',  ( -101.3297067515148200, -284.6404051943337663, -313.1045985470062192 ) ) ;
#86808=CARTESIAN_POINT ( 'NONE',  ( -93.87237594259970308, -285.3694564531878655, -321.6346665297212439 ) ) ;
#86809=CARTESIAN_POINT ( 'NONE',  ( -95.31601251462487312, -284.2003075149974052, -321.0042161784878090 ) ) ;
#86810=CARTESIAN_POINT ( 'NONE',  ( -4.341809925834303918, -280.8328234898870619, -205.2081816685068247 ) ) ;
#86811=CARTESIAN_POINT ( 'NONE',  ( -110.0552246555809290, -267.0563155853889725, -307.0414417294254577 ) ) ;
#86812=CARTESIAN_POINT ( 'NONE',  ( 200.7444845821497381, 293.5020097745142493, -83.02703438293134752 ) ) ;
#86813=CARTESIAN_POINT ( 'NONE',  ( 197.5587112275084394, 287.0354810671433370, -96.43656103357294285 ) ) ;
#86814=CARTESIAN_POINT ( 'NONE',  ( -46.18819073417365217, -273.1342200703788876, -197.7364573587971392 ) ) ;
#86815=CARTESIAN_POINT ( 'NONE',  ( -36.28159082874546471, -294.5468877216721921, -347.3053693379038123 ) ) ;
#86816=CARTESIAN_POINT ( 'NONE',  ( 168.4634583693828347, 229.6213362103191287, -190.1949568163676929 ) ) ;
#86817=CARTESIAN_POINT ( 'NONE',  ( -34.10717456667234870, -272.7768668049313305, -193.9226713860331870 ) ) ;
#86818=CARTESIAN_POINT ( 'NONE',  ( -109.0346373814171841, -298.6633112630831874, -251.0510198752967597 ) ) ;
#86819=CARTESIAN_POINT ( 'NONE',  ( 35.05022486730094755, -288.6974927387190633, -257.3995368237181083 ) ) ;
#86821=CARTESIAN_POINT ( 'NONE',  ( -96.32291540047100398, -296.8302833475544844, -319.5143980008072049 ) ) ;
#86822=CARTESIAN_POINT ( 'NONE',  ( -87.74148201065924013, -285.8169624009063341, -217.4664072097358769 ) ) ;
#86823=CARTESIAN_POINT ( 'NONE',  ( -38.33954403604099781, -272.9602524530000096, -193.6767204910124462 ) ) ;
#86824=CARTESIAN_POINT ( 'NONE',  ( 21.25116090570250904, -295.0264352406897501, -320.0706287109910022 ) ) ;
#86825=CARTESIAN_POINT ( 'NONE',  ( 13.35998917800109531, -294.8576441450132393, -328.3011454666491318 ) ) ;
#86826=CARTESIAN_POINT ( 'NONE',  ( -109.6226499573746764, -290.5828212286703547, -280.6715567784370364 ) ) ;
#86827=ORIENTED_EDGE ( 'NONE', *, *, #47505, .F. ) ;
#86828=CARTESIAN_POINT ( 'NONE',  ( -89.19281939885948418, -275.2500978073297802, -215.3280607889855958 ) ) ;
#86829=CARTESIAN_POINT ( 'NONE',  ( 30.90353918811203116, -273.8966644578293881, -235.5674974730983990 ) ) ;
#86832=CARTESIAN_POINT ( 'NONE',  ( -74.97235823153418721, -279.0724059540298185, -203.2532907640478186 ) ) ;
#86833=CARTESIAN_POINT ( 'NONE',  ( 33.66203403119889970, -274.2157071071154633, -290.5296971300207929 ) ) ;
#86834=CARTESIAN_POINT ( 'NONE',  ( -85.52363296086240041, -274.4472104620744517, -215.0419560849965706 ) ) ;
#86836=CARTESIAN_POINT ( 'NONE',  ( 13.65192824351587397, -275.7295579016390548, -217.7963168958090989 ) ) ;
#86837=CARTESIAN_POINT ( 'NONE',  ( -97.03117657187479494, -274.9495566298397762, -223.3383530757225230 ) ) ;
#86838=CARTESIAN_POINT ( 'NONE',  ( -15.09976078826316304, -274.7857549282261971, -342.4136820837916275 ) ) ;
#86839=CARTESIAN_POINT ( 'NONE',  ( -70.97031699023901297, -296.1595473133397149, -335.2828156419582228 ) ) ;
#86840=CARTESIAN_POINT ( 'NONE',  ( 17.50772934652921009, -292.8232884356419845, -319.4404309214895079 ) ) ;
#86842=CARTESIAN_POINT ( 'NONE',  ( -96.09813322418342807, -278.3745439393069319, -320.0524527527244913 ) ) ;
#86843=CARTESIAN_POINT ( 'NONE',  ( 34.37310310425249327, -275.5389288423594394, -256.7234128284012513 ) ) ;
#86845=CARTESIAN_POINT ( 'NONE',  ( -89.53748335026845950, -284.0200167005681919, -214.3525214772778043 ) ) ;
#86846=CARTESIAN_POINT ( 'NONE',  ( -112.2948881186215857, -298.6331651874568820, -264.0503518517452903 ) ) ;
#86849=CARTESIAN_POINT ( 'NONE',  ( -65.14513454525537384, -284.8766089075410264, -202.6346691717131137 ) ) ;
#86852=CARTESIAN_POINT ( 'NONE',  ( -109.5911086132750114, -277.0016840335301254, -254.2408968133752580 ) ) ;
#86853=CARTESIAN_POINT ( 'NONE',  ( -108.7482153045041002, -276.8933796392527711, -288.2031294237057182 ) ) ;
#86854=CARTESIAN_POINT ( 'NONE',  ( 9.529343247231585323, -284.4081899320830189, -328.9768874560066365 ) ) ;
#86855=CARTESIAN_POINT ( 'NONE',  ( -66.94883841530983659, -278.6541538061674146, -337.5217304590391336 ) ) ;
#86858=CARTESIAN_POINT ( 'NONE',  ( 36.45880250003939693, -274.1919467345923067, -289.3328398162641975 ) ) ;
#86859=CARTESIAN_POINT ( 'NONE',  ( 26.72186456130578236, -275.7220136629193803, -235.0455216226051789 ) ) ;
#86860=CARTESIAN_POINT ( 'NONE',  ( 5.126948894184845784, -282.6251541114432939, -208.3414253479113256 ) ) ;
#86862=CARTESIAN_POINT ( 'NONE',  ( -31.90550056379007415, -290.9043498458780732, -345.7768859654386233 ) ) ;
#86863=CARTESIAN_POINT ( 'NONE',  ( -12.74980523639072949, -290.3715224340365921, -199.4536722586505562 ) ) ;
#86865=CARTESIAN_POINT ( 'NONE',  ( 82.17417184970206279, -297.5662997459467647, -195.6645840736872515 ) ) ;
#86866=CARTESIAN_POINT ( 'NONE',  ( -94.14895943576473769, -271.8932868063695878, -223.7133553978839871 ) ) ;
#86867=CARTESIAN_POINT ( 'NONE',  ( -109.3000413618258193, -288.9291320137709249, -252.0649630799227054 ) ) ;
#86868=CARTESIAN_POINT ( 'NONE',  ( -43.41528170534920861, -158.9639970630164498, -364.8434004397808508 ) ) ;
#86870=CARTESIAN_POINT ( 'NONE',  ( -80.16764853839896432, -288.1000006434949796, -333.5806883127525566 ) ) ;
#86871=CARTESIAN_POINT ( 'NONE',  ( -51.95614118675854343, -284.1075939969323940, -195.7394099293193221 ) ) ;
#86872=CARTESIAN_POINT ( 'NONE',  ( -61.71287943140944776, -284.8002930487787694, -339.8512278002538096 ) ) ;
#86873=EDGE_CURVE ( 'NONE', #8402, #39736, #36994, .T. ) ;
#86874=CARTESIAN_POINT ( 'NONE',  ( -110.4797577696382689, -285.3116262416378390, -273.6555799307682264 ) ) ;
#86875=CARTESIAN_POINT ( 'NONE',  ( -71.45080126392132058, -293.5838877526078932, -203.1532573858007709 ) ) ;
#86876=CARTESIAN_POINT ( 'NONE',  ( -81.24181258839446684, -273.8069192882472862, -207.0626354033265386 ) ) ;
#86877=CARTESIAN_POINT ( 'NONE',  ( -95.45538569605990631, -289.2939843182991808, -222.0491680851177989 ) ) ;
#86878=CARTESIAN_POINT ( 'NONE',  ( -74.09684862173958209, -277.5266836087328102, -338.0374756844877879 ) ) ;
#86879=CARTESIAN_POINT ( 'NONE',  ( 33.10045602775717555, -295.8551362106339866, -295.2091428151940136 ) ) ;
#86880=DIRECTION ( 'NONE',  ( -1.000000000000000000, -0.000000000000000000, -0.000000000000000000 ) ) ;
#86881=CARTESIAN_POINT ( 'NONE',  ( -95.99890600148557951, -299.6948066931273615, -223.6242672951989618 ) ) ;
#86882=CARTESIAN_POINT ( 'NONE',  ( -4.622555397615084161, -281.2965595327100345, -336.1691801607071852 ) ) ;
#86883=CARTESIAN_POINT ( 'NONE',  ( -111.0022715921551111, -276.3593710688597298, -285.3964256195409916 ) ) ;
#86884=CARTESIAN_POINT ( 'NONE',  ( -67.24593133910560994, -272.1469644428377137, -200.1582354957006373 ) ) ;
#86885=CARTESIAN_POINT ( 'NONE',  ( 28.11809138613718773, -275.3427318570775810, -303.0160785147780871 ) ) ;
#86886=CARTESIAN_POINT ( 'NONE',  ( -38.93176445487830506, -293.5519694959696722, -196.6849383197764496 ) ) ;
#86887=CARTESIAN_POINT ( 'NONE',  ( 28.94640993440842180, -294.0727705118734434, -239.1079720788806071 ) ) ;
#86888=CARTESIAN_POINT ( 'NONE',  ( -30.76620544236652677, -293.5588613948452235, -194.1814413712471890 ) ) ;
#86889=CARTESIAN_POINT ( 'NONE',  ( 36.60161389795175069, -294.6192887686886479, -250.6717627220464522 ) ) ;
#86890=CARTESIAN_POINT ( 'NONE',  ( -93.94389333796340225, -295.7327289671717381, -316.4805664725033694 ) ) ;
#86891=CARTESIAN_POINT ( 'NONE',  ( -48.32949609678158964, -291.1920234091790007, -344.6042970538138661 ) ) ;
#86892=CARTESIAN_POINT ( 'NONE',  ( -113.9036362900988451, -284.6162565717947359, -278.5629431221065602 ) ) ;
#86893=CARTESIAN_POINT ( 'NONE',  ( -3.094337321886710956, -272.6392355175495368, -202.7639322579063332 ) ) ;
#86894=CARTESIAN_POINT ( 'NONE',  ( -9.991975442845525635, -286.2327576604603223, -198.3252044889055128 ) ) ;
#86895=CARTESIAN_POINT ( 'NONE',  ( -110.3688160444902309, -280.3326459323677682, -285.8170924691579557 ) ) ;
#86896=CARTESIAN_POINT ( 'NONE',  ( -49.47212374671008916, -284.6891096647627819, -197.9216119406484893 ) ) ;
#86897=CARTESIAN_POINT ( 'NONE',  ( -18.25844294283939817, -286.8060514101995295, -342.8926969051153719 ) ) ;
#86898=CARTESIAN_POINT ( 'NONE',  ( -79.20817858417055390, -277.6337584082548346, -207.1515144517583735 ) ) ;
#86899=CARTESIAN_POINT ( 'NONE',  ( -117.0947446405890418, -269.4376451100752661, -283.8482964293340274 ) ) ;
#86900=CARTESIAN_POINT ( 'NONE',  ( -93.29819437879417876, -284.7263722217711575, -223.3838980455866761 ) ) ;
#86901=CARTESIAN_POINT ( 'NONE',  ( 39.01468303602170806, -282.6800264357202650, -264.2201516214257708 ) ) ;
#86902=CARTESIAN_POINT ( 'NONE',  ( -99.68620203225715670, -289.0152016919855100, -315.1718484472781370 ) ) ;
#86903=CARTESIAN_POINT ( 'NONE',  ( -105.4695610292144607, -280.5972650895556058, -236.1109301535063878 ) ) ;
#86904=CARTESIAN_POINT ( 'NONE',  ( -62.22963551617960576, -278.6842322358107822, -342.7626824613544159 ) ) ;
#86905=CARTESIAN_POINT ( 'NONE',  ( -87.52908431975247083, -279.1615861610893035, -217.2796927199434549 ) ) ;
#86906=CARTESIAN_POINT ( 'NONE',  ( -95.06605684316079419, -275.1878189204332443, -223.0151754470984997 ) ) ;
#86907=CARTESIAN_POINT ( 'NONE',  ( 34.45149188605564206, -293.9047819355489537, -298.1952262028938776 ) ) ;
#86908=CARTESIAN_POINT ( 'NONE',  ( 22.47680562451330744, -286.1852246695798385, -315.0321769504552663 ) ) ;
#86910=CARTESIAN_POINT ( 'NONE',  ( -96.85170157148975534, -292.7964252854051210, -222.7691002997040641 ) ) ;
#86911=CARTESIAN_POINT ( 'NONE',  ( -84.68818116109137861, -294.6426447077963076, -326.3968497534781932 ) ) ;
#86912=CARTESIAN_POINT ( 'NONE',  ( 35.66290118510109153, -293.2601861980901958, -273.4941095296464368 ) ) ;
#86913=CARTESIAN_POINT ( 'NONE',  ( -108.0873074472835924, -292.0099057537805152, -240.7545046334842311 ) ) ;
#86915=CARTESIAN_POINT ( 'NONE',  ( 34.80549816460538892, -282.3586966801141784, -282.1371294821126412 ) ) ;
#86917=CARTESIAN_POINT ( 'NONE',  ( -35.46743192501943298, -296.9954357504116160, -193.6705618249556551 ) ) ;
#86918=CARTESIAN_POINT ( 'NONE',  ( -6.952563875487595801, -289.3151389814750019, -341.0139497990180644 ) ) ;
#86919=CARTESIAN_POINT ( 'NONE',  ( -101.8785350594359755, -282.1645585666854004, -310.0511975511534501 ) ) ;
#86920=CARTESIAN_POINT ( 'NONE',  ( -105.1353412709446786, -290.4138256832785601, -306.8270817300644921 ) ) ;
#86921=CARTESIAN_POINT ( 'NONE',  ( -37.28511670800484978, -286.3861252245957871, -197.3275536068215104 ) ) ;
#86923=CARTESIAN_POINT ( 'NONE',  ( -57.41194557413744093, -168.5696832352114711, -362.2019297073620123 ) ) ;
#86924=CARTESIAN_POINT ( 'NONE',  ( -102.3726955531243732, -253.9557218656232180, -324.0492224005949993 ) ) ;
#86925=CARTESIAN_POINT ( 'NONE',  ( -110.3189945673971692, -277.8176032825532502, -265.1730332779121682 ) ) ;
#86926=CARTESIAN_POINT ( 'NONE',  ( -16.82207620049340946, -279.2438286434855854, -199.9823491192897222 ) ) ;
#86927=CARTESIAN_POINT ( 'NONE',  ( 25.31216207106841765, -274.6260374437338783, -225.6145479451469669 ) ) ;
#86928=CARTESIAN_POINT ( 'NONE',  ( 195.1835355330036066, 276.0653920892696647, -124.6905694975844909 ) ) ;
#86929=CARTESIAN_POINT ( 'NONE',  ( -38.14536149072925042, -278.6169999800464439, -193.9545709877129411 ) ) ;
#86930=CARTESIAN_POINT ( 'NONE',  ( -18.34075180822417295, -280.8263642058910818, -342.6006431026112864 ) ) ;
#86931=CARTESIAN_POINT ( 'NONE',  ( 8.315406922725703254, -296.1969989576587636, -331.1015706242496890 ) ) ;
#86932=CIRCLE ( 'NONE', #80850, 1.895975569037589015 ) ;
#86933=CARTESIAN_POINT ( 'NONE',  ( -65.35634990667689692, -292.1681717458145044, -202.8704265452473692 ) ) ;
#86934=CARTESIAN_POINT ( 'NONE',  ( -5.594463263340846204, -287.3103928393369983, -336.6435170880935743 ) ) ;
#86935=CARTESIAN_POINT ( 'NONE',  ( 35.63059290751954933, -275.8959179690296537, -245.9372457096550875 ) ) ;
#86936=CARTESIAN_POINT ( 'NONE',  ( -100.1653902561143212, -296.2067918880113666, -307.6383807713285705 ) ) ;
#86940=CARTESIAN_POINT ( 'NONE',  ( -73.10605034128096236, -281.5020973758564082, -203.7865058852713105 ) ) ;
#86941=CARTESIAN_POINT ( 'NONE',  ( 22.35726285581571204, -282.0399586273710497, -227.8139689271587827 ) ) ;
#86942=CARTESIAN_POINT ( 'NONE',  ( -83.96311874118413243, -281.1821475650824596, -210.2910391935556049 ) ) ;
#86943=CARTESIAN_POINT ( 'NONE',  ( 35.92305283820380168, -280.5876029057382652, -268.5898071631148696 ) ) ;
#86944=CARTESIAN_POINT ( 'NONE',  ( -31.26340798893588513, -272.6101549384391092, -196.9061115795442163 ) ) ;
#86947=CARTESIAN_POINT ( 'NONE',  ( 39.46250208819142813, -276.4009146000140618, -274.0260451032287392 ) ) ;
#86949=CARTESIAN_POINT ( 'NONE',  ( 34.65847069133043590, -277.2798301904471145, -249.1804188694425477 ) ) ;
#86950=CARTESIAN_POINT ( 'NONE',  ( -99.18364715087494687, -276.5266253956545484, -315.2629889391303095 ) ) ;
#86952=LINE ( 'NONE', #88345, #83717 ) ;
#86953=CARTESIAN_POINT ( 'NONE',  ( -101.5040988635992960, -286.0042478258033043, -309.8781192586051816 ) ) ;
#86954=CARTESIAN_POINT ( 'NONE',  ( 2.336642849746430883, -291.7955606787663783, -208.8337853208038553 ) ) ;
#86955=CARTESIAN_POINT ( 'NONE',  ( -26.62709092398780797, -285.5334963370459036, -194.1597417034820126 ) ) ;
#86956=CARTESIAN_POINT ( 'NONE',  ( -32.09594336733599107, -281.2249262236850313, -344.1883219797156244 ) ) ;
#86957=CARTESIAN_POINT ( 'NONE',  ( -93.01672211941095725, -282.4465694361184092, -318.5016762859595474 ) ) ;
#86958=CARTESIAN_POINT ( 'NONE',  ( -53.76366360659341126, -284.4725734779144091, -341.9498346190770235 ) ) ;
#86959=CARTESIAN_POINT ( 'NONE',  ( -64.16049008565703105, -271.7021451119229027, -200.3062209477518252 ) ) ;
#86960=CARTESIAN_POINT ( 'NONE',  ( -108.2762202343852493, -283.3101978162937939, -242.3836714580931186 ) ) ;
#86961=CARTESIAN_POINT ( 'NONE',  ( -85.10161127984252971, -297.7116797439952620, -328.1883739475700281 ) ) ;
#86962=CARTESIAN_POINT ( 'NONE',  ( -103.5877890818818940, -279.9153425415879042, -239.0190653664648153 ) ) ;
#86963=CARTESIAN_POINT ( 'NONE',  ( -112.3250561810371124, -286.6284405422214263, -264.4191461670728245 ) ) ;
#86966=CARTESIAN_POINT ( 'NONE',  ( 33.11112878676183868, -295.1180981235899594, -242.9088996363635147 ) ) ;
#86967=CARTESIAN_POINT ( 'NONE',  ( -37.84814670879880794, -275.0583030136047000, -345.3722060482741085 ) ) ;
#86968=CARTESIAN_POINT ( 'NONE',  ( 18.52038806274003946, -287.4713679625443206, -323.1208177864992876 ) ) ;
#86969=CARTESIAN_POINT ( 'NONE',  ( 33.10444211210852217, -292.2403355145663113, -292.3561505787731676 ) ) ;
#86970=CARTESIAN_POINT ( 'NONE',  ( -43.26340984704629022, -275.8133174678249588, -343.6153112563832792 ) ) ;
#86971=CARTESIAN_POINT ( 'NONE',  ( -110.3613397655482800, -294.5172644084547642, -283.8106600007712927 ) ) ;
#86972=CARTESIAN_POINT ( 'NONE',  ( -90.18245116389111615, -292.6004517020554090, -219.2817825534721123 ) ) ;
#86973=CARTESIAN_POINT ( 'NONE',  ( -95.99890600148557951, -275.6948066931273615, -223.6242672951989618 ) ) ;
#86974=CARTESIAN_POINT ( 'NONE',  ( -65.36703677767771126, -293.8917826647602851, -341.3490696980040866 ) ) ;
#86975=CARTESIAN_POINT ( 'NONE',  ( -26.33567588664358894, -290.5100280659751206, -343.3874350281475358 ) ) ;
#86976=CARTESIAN_POINT ( 'NONE',  ( -110.2534416265384465, -289.0639868653782969, -248.9636422866416581 ) ) ;
#86977=CARTESIAN_POINT ( 'NONE',  ( 34.86582325785120418, -289.1640144951885532, -284.6195935761369356 ) ) ;
#86980=CARTESIAN_POINT ( 'NONE',  ( -45.37003679551985869, -289.9593068960140840, -343.0807682649054300 ) ) ;
#86982=CARTESIAN_POINT ( 'NONE',  ( -82.60560315862981895, -290.8605763411180192, -332.1606956507961286 ) ) ;
#86983=CARTESIAN_POINT ( 'NONE',  ( -98.08669643901508550, -277.1776928089325338, -225.7472852597653343 ) ) ;
#86984=CARTESIAN_POINT ( 'NONE',  ( -98.56212380429246878, -279.5079335254365560, -223.6726962794251676 ) ) ;
#86985=CARTESIAN_POINT ( 'NONE',  ( -1.647712679428733340, -282.2588758213220217, -338.5643697497121138 ) ) ;
#86986=CARTESIAN_POINT ( 'NONE',  ( 35.64158622496402273, -285.7738233004019435, -287.6365504340372468 ) ) ;
#86988=CARTESIAN_POINT ( 'NONE',  ( 36.26061997301022899, -279.5612842513538112, -260.3051696439986813 ) ) ;
#86989=CARTESIAN_POINT ( 'NONE',  ( -62.50577743955250298, -283.7245651208776849, -199.7086597029409347 ) ) ;
#86990=CARTESIAN_POINT ( 'NONE',  ( 193.8404911864852807, 275.6304217925664375, -124.1201752808129868 ) ) ;
#86991=CARTESIAN_POINT ( 'NONE',  ( -112.3873194491561947, -276.8567785726466468, -284.2483146577494608 ) ) ;
#86993=CARTESIAN_POINT ( 'NONE',  ( -112.2262514165583980, -283.2647117677900042, -286.9079149419546866 ) ) ;
#86994=CARTESIAN_POINT ( 'NONE',  ( -94.74575753952395019, -273.9936287187117614, -225.0028120148074890 ) ) ;
#86995=CARTESIAN_POINT ( 'NONE',  ( -57.89709525034378146, -293.3824679963095150, -199.4280681820043242 ) ) ;
#86996=CARTESIAN_POINT ( 'NONE',  ( 7.611735474325791451, -299.9190521943205567, -193.8444490797695892 ) ) ;
#86997=CARTESIAN_POINT ( 'NONE',  ( 35.37467869294165723, -275.3067595654924276, -277.0256313092192499 ) ) ;
#86998=CARTESIAN_POINT ( 'NONE',  ( -66.81629585481445588, -297.4385148196970476, -339.3266808211263310 ) ) ;
#86999=CARTESIAN_POINT ( 'NONE',  ( -51.68322501210588626, -289.3974450965746996, -346.0137495857400722 ) ) ;
#87000=CARTESIAN_POINT ( 'NONE',  ( 23.92507970797107930, -280.2298337478353574, -314.6063225004766082 ) ) ;
#87001=CARTESIAN_POINT ( 'NONE',  ( 6.497972222874298431, -292.4633888009562952, -207.0595924665827852 ) ) ;
#87002=CARTESIAN_POINT ( 'NONE',  ( -102.6138556948706508, -290.0618516025776330, -237.0381423371707967 ) ) ;
#87003=CARTESIAN_POINT ( 'NONE',  ( 24.83897527482761447, -292.1192734703168412, -312.2963568091732895 ) ) ;
#87006=CARTESIAN_POINT ( 'NONE',  ( -104.7574332432651829, -290.4388306379360642, -242.0673282533112456 ) ) ;
#87008=CARTESIAN_POINT ( 'NONE',  ( -2.340916204399413392, -287.4450511932226391, -202.0253653276260479 ) ) ;
#87009=CARTESIAN_POINT ( 'NONE',  ( -109.1418805571601069, -299.0519495502701943, -270.3937649182068412 ) ) ;
#87010=CARTESIAN_POINT ( 'NONE',  ( 17.38536455716302598, -293.3529204309299416, -324.2676370243960378 ) ) ;
#87011=CARTESIAN_POINT ( 'NONE',  ( -94.02246708635550476, -285.1645415923574092, -321.7672042702283761 ) ) ;
#87012=CARTESIAN_POINT ( 'NONE',  ( -69.98052506961970209, -285.4431632047923699, -205.0501058414645001 ) ) ;
#87013=CARTESIAN_POINT ( 'NONE',  ( 34.57409704039786646, -277.2832580352981040, -286.5066311276393662 ) ) ;
#87014=CARTESIAN_POINT ( 'NONE',  ( -2.395542853222797142, -292.6074731187071620, -336.3202939689280129 ) ) ;
#87015=CARTESIAN_POINT ( 'NONE',  ( 26.68028261265103396, -295.8147902596743961, -307.4981579518927788 ) ) ;
#87016=CARTESIAN_POINT ( 'NONE',  ( 17.72301747027863783, -275.0365047420391988, -318.9084919940676741 ) ) ;
#87019=CARTESIAN_POINT ( 'NONE',  ( -47.63294801514003751, -294.8463092448595262, -346.6489578287052495 ) ) ;
#87020=CARTESIAN_POINT ( 'NONE',  ( 22.34241534179654209, -290.0846403591799572, -314.8697723763079352 ) ) ;
#87021=CARTESIAN_POINT ( 'NONE',  ( 201.1758259809593596, 294.8492306316788927, -54.00000000001604405 ) ) ;
#87022=CARTESIAN_POINT ( 'NONE',  ( -110.5007710126116365, -297.3410710553436047, -293.4103266072941096 ) ) ;
#87023=CARTESIAN_POINT ( 'NONE',  ( 31.93455021491516632, -287.8939574015018934, -247.0224417871119726 ) ) ;
#87024=CARTESIAN_POINT ( 'NONE',  ( -111.5006029407103370, -277.8605462609007759, -250.4791783278814705 ) ) ;
#87025=CARTESIAN_POINT ( 'NONE',  ( -41.93117385229657401, -295.7598318103241013, -347.1744318594986112 ) ) ;
#87026=CARTESIAN_POINT ( 'NONE',  ( -84.41606186059408401, -287.8313947895858860, -329.7939702951457548 ) ) ;
#87027=CARTESIAN_POINT ( 'NONE',  ( -108.3538937382227516, -296.5058244838007226, -300.2145888350063387 ) ) ;
#87030=CARTESIAN_POINT ( 'NONE',  ( 189.4028190526519779, 267.9912538632855785, -137.5853595571369965 ) ) ;
#87031=CARTESIAN_POINT ( 'NONE',  ( -21.15012816928218697, -287.7763675391628908, -195.7920845411168216 ) ) ;
#87032=CARTESIAN_POINT ( 'NONE',  ( 36.60358173371529489, -290.6237833571632905, -234.7871824221999191 ) ) ;
#87033=ORIENTED_EDGE ( 'NONE', *, *, #87263, .F. ) ;
#87035=CARTESIAN_POINT ( 'NONE',  ( -112.8944733477863309, -278.0809647510012610, -255.9697284346143533 ) ) ;
#87036=CARTESIAN_POINT ( 'NONE',  ( -95.69909136722677090, -285.9062825057794726, -317.2263788409240419 ) ) ;
#87038=CARTESIAN_POINT ( 'NONE',  ( -97.10808725633442862, -283.7692305905869716, -222.7524500176436391 ) ) ;
#87039=CARTESIAN_POINT ( 'NONE',  ( -73.07109516919334169, -287.6094922979007720, -335.6659763733678687 ) ) ;
#87040=CARTESIAN_POINT ( 'NONE',  ( 23.39194428265797043, -278.0249123827697417, -315.6571434105271123 ) ) ;
#87041=CARTESIAN_POINT ( 'NONE',  ( -108.9437786015251817, -296.8521621837246585, -284.9537369827323232 ) ) ;
#87043=CARTESIAN_POINT ( 'NONE',  ( -67.51287524442672350, -294.1412501299630549, -337.3894218181170004 ) ) ;
#87044=CARTESIAN_POINT ( 'NONE',  ( -22.59386719112204034, -280.8874469842747317, -194.8363170886761111 ) ) ;
#87045=CARTESIAN_POINT ( 'NONE',  ( -110.3511811492682284, -278.5845093988793337, -267.9082630551762918 ) ) ;
#87046=CARTESIAN_POINT ( 'NONE',  ( -79.10631899854433868, -278.8205096865286805, -210.3643740832142726 ) ) ;
#87047=CARTESIAN_POINT ( 'NONE',  ( 11.57790059813620509, -275.7919959780149384, -211.2297373291249869 ) ) ;
#87048=CARTESIAN_POINT ( 'NONE',  ( -28.64978108595942530, -275.8648454504322558, -346.6112166353418615 ) ) ;
#87050=CARTESIAN_POINT ( 'NONE',  ( -54.27093570039709647, -275.2692864570307734, -343.4781719471016004 ) ) ;
#87051=CARTESIAN_POINT ( 'NONE',  ( -106.6244182717853448, -297.5617832728611916, -302.5870587432296475 ) ) ;
#87052=CARTESIAN_POINT ( 'NONE',  ( 35.78497577281001440, -278.2662352645559167, -287.0191576251351080 ) ) ;
#87053=CARTESIAN_POINT ( 'NONE',  ( -47.20788896421541381, -156.8319029772612225, -362.3615984655540387 ) ) ;
#87054=CARTESIAN_POINT ( 'NONE',  ( -27.80991693150940591, -287.2557188261831698, -197.6743160014825946 ) ) ;
#87055=CARTESIAN_POINT ( 'NONE',  ( -57.50885758819714511, -287.5555889590203265, -197.0449057537632598 ) ) ;
#87056=CARTESIAN_POINT ( 'NONE',  ( 33.17803229305736323, -287.1570333691416295, -289.8066071122917720 ) ) ;
#87057=CARTESIAN_POINT ( 'NONE',  ( -111.0802993045079319, -276.9127413090307641, -273.3710024826641529 ) ) ;
#87058=CARTESIAN_POINT ( 'NONE',  ( -104.6146896406658016, -286.8307805137546893, -238.8511167778089828 ) ) ;
#87059=CARTESIAN_POINT ( 'NONE',  ( -108.2805216480688415, -277.2939342212549718, -250.3546492497199552 ) ) ;
#87060=CARTESIAN_POINT ( 'NONE',  ( -11.06216349228297879, -278.0174523273245200, -338.9951433077949332 ) ) ;
#87061=CARTESIAN_POINT ( 'NONE',  ( 15.48695484835621272, -275.3164036159712964, -219.8188731429957556 ) ) ;
#87062=CARTESIAN_POINT ( 'NONE',  ( 39.20672379671495378, -286.3980690455695708, -274.4172908513317566 ) ) ;
#87064=CARTESIAN_POINT ( 'NONE',  ( 31.87156146139217583, -281.9245724303455063, -236.8668499724868184 ) ) ;
#87065=CARTESIAN_POINT ( 'NONE',  ( 37.48998451762362549, -282.2689636264242381, -288.2987734089523997 ) ) ;
#87069=CARTESIAN_POINT ( 'NONE',  ( -12.60427254789684604, -290.5944431088615261, -342.0287051547421697 ) ) ;
#87070=CARTESIAN_POINT ( 'NONE',  ( -80.27779731921161499, -288.3049155917591975, -333.7480283163351373 ) ) ;
#87071=CARTESIAN_POINT ( 'NONE',  ( -71.69494316103349263, -297.0986235452331243, -338.3779917053607846 ) ) ;
#87072=CARTESIAN_POINT ( 'NONE',  ( -93.08511059206676919, -272.2845389004573917, -222.8435468249676887 ) ) ;
#87073=CARTESIAN_POINT ( 'NONE',  ( -13.88963751095280408, -291.6971190372616434, -197.0705678946828243 ) ) ;
#87074=CARTESIAN_POINT ( 'NONE',  ( 35.25378180290265817, -285.8626547997351963, -257.3998924987257055 ) ) ;
#87075=CARTESIAN_POINT ( 'NONE',  ( -41.62943686792771558, -290.2374042891395902, -196.4215450113670443 ) ) ;
#87076=CARTESIAN_POINT ( 'NONE',  ( 24.58153917179780024, -289.2990844575876963, -309.7647084178387900 ) ) ;
#87077=CARTESIAN_POINT ( 'NONE',  ( -95.95921662488163406, -292.4090924074130839, -317.1477375740089997 ) ) ;
#87078=CARTESIAN_POINT ( 'NONE',  ( 27.19604713815770225, -290.0633536425456214, -308.5694917326212590 ) ) ;
#87079=CARTESIAN_POINT ( 'NONE',  ( -110.2108464810266071, -288.7889813426107253, -251.8671125422930004 ) ) ;
#87080=CARTESIAN_POINT ( 'NONE',  ( 15.19916572695814949, -294.7935788443522824, -216.7692228310467328 ) ) ;
#87081=CARTESIAN_POINT ( 'NONE',  ( -109.6553682008042472, -285.6467479481958094, -258.6996405168739557 ) ) ;
#87082=CARTESIAN_POINT ( 'NONE',  ( 37.03396929114710190, -295.4085114556111193, -259.1366410626119432 ) ) ;
#87083=CARTESIAN_POINT ( 'NONE',  ( -114.2951601902143608, -272.0832046287694652, -270.3551471570179956 ) ) ;
#87085=CARTESIAN_POINT ( 'NONE',  ( -26.49281569206767628, -300.1071026503124131, -194.7975931931764535 ) ) ;
#87086=CARTESIAN_POINT ( 'NONE',  ( 31.50307961130697976, -281.0801043631039988, -295.2696458960037944 ) ) ;
#87087=CARTESIAN_POINT ( 'NONE',  ( -45.89210104889916408, -281.1602700858851449, -344.9245251598084110 ) ) ;
#87088=CARTESIAN_POINT ( 'NONE',  ( -114.0732210017862798, -295.6871888938720190, -275.3187444137123521 ) ) ;
#87089=CARTESIAN_POINT ( 'NONE',  ( -4.843157671766616268, -272.7259712287394677, -203.8503419411900097 ) ) ;
#87090=CARTESIAN_POINT ( 'NONE',  ( -62.29512720161778105, -275.4589498511286365, -340.5489471361688629 ) ) ;
#87091=CARTESIAN_POINT ( 'NONE',  ( -95.69075116023063288, -298.4919283886091534, -225.6569217723902625 ) ) ;
#87092=CARTESIAN_POINT ( 'NONE',  ( -43.97339029149914325, -272.5447403110272830, -194.1857708260686195 ) ) ;
#87093=CARTESIAN_POINT ( 'NONE',  ( -113.3531685960080608, -294.7659223054623112, -272.4196762500802720 ) ) ;
#87094=CARTESIAN_POINT ( 'NONE',  ( -31.53792181364288538, -296.4028650608722728, -343.7716455480905893 ) ) ;
#87096=CARTESIAN_POINT ( 'NONE',  ( -73.37304601109943292, -296.3460879544666113, -334.0348475812049287 ) ) ;
#87098=CARTESIAN_POINT ( 'NONE',  ( -96.27787509257909448, -283.2147005265668440, -223.4043922827694075 ) ) ;
#87099=CARTESIAN_POINT ( 'NONE',  ( -88.12574357754172638, -297.3174204619543843, -217.8502831476394022 ) ) ;
#87100=CARTESIAN_POINT ( 'NONE',  ( -111.8749650846900607, -284.3095831587860403, -289.7471031355258901 ) ) ;
#87101=CARTESIAN_POINT ( 'NONE',  ( 23.11786949616666220, -284.0869466274041315, -315.6816943435726444 ) ) ;
#87102=CARTESIAN_POINT ( 'NONE',  ( 31.40481746806630170, -286.7730608759853226, -235.7250008526249019 ) ) ;
#87103=CARTESIAN_POINT ( 'NONE',  ( 30.40890565665472778, -291.1318313133708671, -238.4600631311398615 ) ) ;
#87104=CARTESIAN_POINT ( 'NONE',  ( -111.1792401077926655, -278.0164947493470891, -249.0966755861460342 ) ) ;
#87105=CARTESIAN_POINT ( 'NONE',  ( -69.85430415644619018, -271.1237833571632905, -202.7746430608542312 ) ) ;
#87106=CARTESIAN_POINT ( 'NONE',  ( 120.8395553409046528, -299.5541904835127980, -195.3611179825600175 ) ) ;
#87107=CARTESIAN_POINT ( 'NONE',  ( 33.77710695988081824, -286.1082654230667117, -252.1652155683320018 ) ) ;
#87108=CARTESIAN_POINT ( 'NONE',  ( -113.9432164640101774, -289.4260050711258145, -274.0624966428848666 ) ) ;
#87111=CARTESIAN_POINT ( 'NONE',  ( -77.48974504741970293, -279.0045281773539045, -335.4359859423503849 ) ) ;
#87112=CARTESIAN_POINT ( 'NONE',  ( -110.3807832951234644, -294.3346195551673645, -288.9524052189986492 ) ) ;
#87113=CARTESIAN_POINT ( 'NONE',  ( 19.36577322110076338, -281.8698058694361634, -316.3846295146207694 ) ) ;
#87114=CARTESIAN_POINT ( 'NONE',  ( -30.58883720292238451, -295.1356695334509368, -347.0644350348135845 ) ) ;
#87115=CARTESIAN_POINT ( 'NONE',  ( -97.83034029730403347, -281.1571022390884309, -225.9984249545709076 ) ) ;
#87116=CARTESIAN_POINT ( 'NONE',  ( -110.4772675662958505, -295.5606560976330570, -274.1817492113691515 ) ) ;
#87119=CARTESIAN_POINT ( 'NONE',  ( -5.304633972890733240, -284.6084617901147453, -337.7953044748188063 ) ) ;
#87121=CARTESIAN_POINT ( 'NONE',  ( -37.30987171927208834, -295.5523547857347353, -195.3611179825600175 ) ) ;
#87122=CARTESIAN_POINT ( 'NONE',  ( -36.93030901808022293, -273.2543841515934560, -193.5106700426319435 ) ) ;
#87123=CARTESIAN_POINT ( 'NONE',  ( -109.7897746165363912, -290.2672776954267420, -279.3208337936673615 ) ) ;
#87124=CARTESIAN_POINT ( 'NONE',  ( 19.35726196656250764, -282.4107136871275543, -223.2678162970068456 ) ) ;
#87126=CARTESIAN_POINT ( 'NONE',  ( 17.87065506638449364, -276.4593907467981353, -221.3156728368727215 ) ) ;
#87127=CARTESIAN_POINT ( 'NONE',  ( -30.26865301048117729, -284.5642067740689072, -346.2321428832173069 ) ) ;
#87128=CARTESIAN_POINT ( 'NONE',  ( 35.42854188223928702, -280.2165187571731053, -260.4106963311598406 ) ) ;
#87129=CARTESIAN_POINT ( 'NONE',  ( -96.38059613480717758, -281.1872334106495828, -224.0866872121109736 ) ) ;
#87130=CARTESIAN_POINT ( 'NONE',  ( -23.35982626625671088, -298.2226792870364989, -193.3611167184400017 ) ) ;
#87131=CARTESIAN_POINT ( 'NONE',  ( 18.09107174954792185, -274.6530169926743952, -216.8410750332150201 ) ) ;
#87132=CARTESIAN_POINT ( 'NONE',  ( -2.447522372816185676, -296.5068889811529971, -336.1160460021952758 ) ) ;
#87135=CARTESIAN_POINT ( 'NONE',  ( -50.28027257718496656, -293.3550626916551209, -345.0660504698409454 ) ) ;
#87136=CARTESIAN_POINT ( 'NONE',  ( -87.37087880576848420, -272.8395320939962403, -217.0464830100559652 ) ) ;
#87137=CARTESIAN_POINT ( 'NONE',  ( -47.66889549982923313, -293.4433888506345625, -194.7031979721988932 ) ) ;
#87138=CARTESIAN_POINT ( 'NONE',  ( 10.64812456238590066, -278.9090924074130839, -330.4860931364851808 ) ) ;
#87139=CARTESIAN_POINT ( 'NONE',  ( 23.64972068570362751, -294.1361410877461253, -223.9924203886815803 ) ) ;
#87140=EDGE_CURVE ( 'NONE', #49115, #34721, #22756, .T. ) ;
#87141=CARTESIAN_POINT ( 'NONE',  ( 23.46592035992629377, -290.1470718755962253, -313.9783361296704811 ) ) ;
#87142=CARTESIAN_POINT ( 'NONE',  ( 35.67666471611626378, -273.7635456059043122, -286.8005948857149860 ) ) ;
#87143=CARTESIAN_POINT ( 'NONE',  ( -54.25785754193617549, -279.1911149806169874, -342.9067508370486621 ) ) ;
#87144=CARTESIAN_POINT ( 'NONE',  ( 31.91651186019259256, -291.9915118503744793, -297.7896536970665693 ) ) ;
#87145=CARTESIAN_POINT ( 'NONE',  ( 25.70735001552274923, -283.9745544798616379, -312.3744820030636902 ) ) ;
#87147=CARTESIAN_POINT ( 'NONE',  ( -45.64608678021451027, -282.8268807630514061, -342.9595229892038901 ) ) ;
#87148=CARTESIAN_POINT ( 'NONE',  ( -35.35785991662786643, -281.1561399079281500, -193.6828076952699291 ) ) ;
#87149=CARTESIAN_POINT ( 'NONE',  ( -78.95694937922455381, -282.3948665894953933, -334.6742562024286940 ) ) ;
#87150=CARTESIAN_POINT ( 'NONE',  ( -9.286615870786235405, -277.6354584490172783, -341.8155262461882558 ) ) ;
#87152=CARTESIAN_POINT ( 'NONE',  ( 18.40998617398158288, -277.7892767476644735, -322.4615712163483749 ) ) ;
#87154=CARTESIAN_POINT ( 'NONE',  ( 30.91033621190086578, -290.2662352645559167, -285.9065529553535612 ) ) ;
#87156=CARTESIAN_POINT ( 'NONE',  ( -96.89220901608568681, -299.1768040567841354, -224.7470093052217521 ) ) ;
#87157=CARTESIAN_POINT ( 'NONE',  ( -96.59368509299753214, -275.9476666652178096, -315.7598964236245251 ) ) ;
#87158=CARTESIAN_POINT ( 'NONE',  ( -70.47635915819078889, -293.3814465750955947, -201.9793339401152252 ) ) ;
#87159=CARTESIAN_POINT ( 'NONE',  ( 6.116887529115544453, -293.7935981579256577, -329.2055190867316128 ) ) ;
#87160=CARTESIAN_POINT ( 'NONE',  ( 27.38962620700064576, -287.6069102190861031, -312.0451817811361366 ) ) ;
#87162=CARTESIAN_POINT ( 'NONE',  ( -50.38493665318376458, -293.7901362928752746, -345.7039622598906590 ) ) ;
#87163=CARTESIAN_POINT ( 'NONE',  ( -108.8736165782340208, -282.7149901221792447, -288.5167051683990849 ) ) ;
#87164=CARTESIAN_POINT ( 'NONE',  ( -50.95511739685161245, -291.0882253555936927, -343.3899680524128826 ) ) ;
#87165=CARTESIAN_POINT ( 'NONE',  ( -77.40995748873682203, -283.9842074098854710, -208.4520365991952247 ) ) ;
#87166=CARTESIAN_POINT ( 'NONE',  ( -36.16897720810293038, -284.3523203412029261, -343.8449134781333214 ) ) ;
#87167=CARTESIAN_POINT ( 'NONE',  ( -98.83344105714425609, -290.8799114488745090, -316.3348478844704346 ) ) ;
#87168=CARTESIAN_POINT ( 'NONE',  ( 30.07586868192587204, -281.6670994347393275, -242.2033507195215520 ) ) ;
#87169=CARTESIAN_POINT ( 'NONE',  ( -37.70258949093786782, -293.8514716091232231, -346.9762075267503860 ) ) ;
#87170=CARTESIAN_POINT ( 'NONE',  ( 3.103851776506648896, -289.3268164014589274, -335.7558910395454745 ) ) ;
#87171=CARTESIAN_POINT ( 'NONE',  ( 35.89110286209584189, -288.3413872990493587, -293.9510198350824908 ) ) ;
#87172=CARTESIAN_POINT ( 'NONE',  ( -85.72773610322461479, -285.5270718311205087, -215.6328594001012959 ) ) ;
#87173=ORIENTED_EDGE ( 'NONE', *, *, #37333, .T. ) ;
#87175=CARTESIAN_POINT ( 'NONE',  ( 22.21565044364082553, -296.0492245353190697, -317.2138473581729272 ) ) ;
#87176=CARTESIAN_POINT ( 'NONE',  ( -58.72962035045954821, -294.0078287156442229, -343.8728224411968881 ) ) ;
#87177=CARTESIAN_POINT ( 'NONE',  ( -102.0704635766277022, -277.1457623696255155, -304.6189000161161857 ) ) ;
#87178=CARTESIAN_POINT ( 'NONE',  ( -66.19831783440207573, -273.1920785887881493, -199.0249959068005126 ) ) ;
#87179=CARTESIAN_POINT ( 'NONE',  ( 6.459642732922678654, -292.9250292024290161, -329.6880967489092882 ) ) ;
#87180=CARTESIAN_POINT ( 'NONE',  ( 14.18629278656914749, -276.5483151905087880, -217.2307127665802113 ) ) ;
#87181=CARTESIAN_POINT ( 'NONE',  ( -63.72391872432801563, -271.8441288913015796, -200.9583209718786350 ) ) ;
#87182=CARTESIAN_POINT ( 'NONE',  ( 20.84734080478926188, -295.3835978332341483, -315.1160951734532318 ) ) ;
#87183=CARTESIAN_POINT ( 'NONE',  ( 35.01683525324736479, -294.4762225124824795, -258.5154492406280156 ) ) ;
#87185=CARTESIAN_POINT ( 'NONE',  ( -109.0561248548955149, -294.8438361494001470, -247.6705587521980192 ) ) ;
#87186=CARTESIAN_POINT ( 'NONE',  ( -109.9526215170702983, -273.6725390570174454, -245.2252289925691002 ) ) ;
#87187=CARTESIAN_POINT ( 'NONE',  ( -42.66910236538571866, -290.0621225498153422, -343.4531556601870648 ) ) ;
#87188=CARTESIAN_POINT ( 'NONE',  ( -93.95624647803359153, -296.2326091545078839, -316.4988844709282034 ) ) ;
#87189=CARTESIAN_POINT ( 'NONE',  ( -110.5706760458231486, -280.3042047991052073, -288.1893392489516827 ) ) ;
#87190=CARTESIAN_POINT ( 'NONE',  ( -112.3137577669544243, -277.0442467264654169, -285.6735146127546159 ) ) ;
#87191=CARTESIAN_POINT ( 'NONE',  ( 11.42154817797827704, -281.7452453484582406, -329.8897384340091321 ) ) ;
#87192=CARTESIAN_POINT ( 'NONE',  ( 13.90273716865263864, -274.0970986852495912, -212.9547943688261569 ) ) ;
#87193=CARTESIAN_POINT ( 'NONE',  ( -45.82743490355252902, -281.2402636095860089, -344.3678791785675344 ) ) ;
#87194=CARTESIAN_POINT ( 'NONE',  ( -104.0829795028111135, -277.4333052205451509, -233.5909936821545330 ) ) ;
#87195=CARTESIAN_POINT ( 'NONE',  ( 2.863406806513552727, -278.5897569061328909, -206.7891693712074925 ) ) ;
#87196=CARTESIAN_POINT ( 'NONE',  ( -80.00078017821981291, -296.1460110460122905, -210.5159313249120601 ) ) ;
#87197=CARTESIAN_POINT ( 'NONE',  ( -4.295077914976588751, -276.4878083470302386, -203.0201134692841833 ) ) ;
#87199=CARTESIAN_POINT ( 'NONE',  ( -37.76004497004281291, -290.0670494313489485, -195.0070749915740009 ) ) ;
#87200=CARTESIAN_POINT ( 'NONE',  ( -43.18229547018431447, -289.1239828260511331, -347.1392883570213144 ) ) ;
#87201=CARTESIAN_POINT ( 'NONE',  ( 12.72392577116737655, -276.7482455560452195, -214.2250033927584241 ) ) ;
#87202=CARTESIAN_POINT ( 'NONE',  ( -61.07376076949173438, -295.7433451161675180, -199.3357716021132262 ) ) ;
#87203=CARTESIAN_POINT ( 'NONE',  ( -111.7212414572205716, -283.5068803817931666, -289.6965311120846422 ) ) ;
#87205=CARTESIAN_POINT ( 'NONE',  ( -74.34580869418557825, -283.5600276426087021, -205.1107906316208016 ) ) ;
#87206=CARTESIAN_POINT ( 'NONE',  ( -114.0438498160389287, -273.6021560138187851, -270.3744733279939965 ) ) ;
#87207=CARTESIAN_POINT ( 'NONE',  ( 0.1248664753035984842, -291.3579588099480588, -207.2470395860473218 ) ) ;
#87208=CARTESIAN_POINT ( 'NONE',  ( -44.11386370735301909, -284.1051911836536306, -196.4354574813377781 ) ) ;
#87211=CARTESIAN_POINT ( 'NONE',  ( 20.91498251029369726, -290.9013635880187962, -223.1056449038877929 ) ) ;
#87212=CARTESIAN_POINT ( 'NONE',  ( -68.91738896012196847, -281.9396976273079076, -339.8425449067846102 ) ) ;
#87213=CARTESIAN_POINT ( 'NONE',  ( -10.94911688531545302, -278.3023607232528889, -339.2804328735938952 ) ) ;
#87214=CARTESIAN_POINT ( 'NONE',  ( -73.43954003664197216, -286.7896081581682779, -202.7379149654411208 ) ) ;
#87215=CARTESIAN_POINT ( 'NONE',  ( -108.6649057187028404, -284.7581362593735435, -254.7463981876746857 ) ) ;
#87217=CARTESIAN_POINT ( 'NONE',  ( -43.23633775017284364, -278.5533215880736861, -343.7138831971363970 ) ) ;
#87218=CARTESIAN_POINT ( 'NONE',  ( -92.33656088284212160, -280.0423235944534781, -222.0909738850105839 ) ) ;
#87219=CARTESIAN_POINT ( 'NONE',  ( -97.74894308766454287, -287.1595758922238701, -225.8237952280231866 ) ) ;
#87222=CARTESIAN_POINT ( 'NONE',  ( -113.7745233062622674, -296.5021401980130804, -261.0324768428683342 ) ) ;
#87223=CARTESIAN_POINT ( 'NONE',  ( 32.02277743232583163, -289.8944956478781592, -298.0762873916737021 ) ) ;
#87225=CARTESIAN_POINT ( 'NONE',  ( 25.22466315766300227, -284.6948066931273047, -320.2154176792147382 ) ) ;
#87226=CARTESIAN_POINT ( 'NONE',  ( -111.8780292072525668, -277.2451370597510163, -288.4668726249474844 ) ) ;
#87227=CARTESIAN_POINT ( 'NONE',  ( 18.83975353840251898, -291.2443608084994366, -218.8821448026533858 ) ) ;
#87228=CARTESIAN_POINT ( 'NONE',  ( 35.68048966333870453, -288.9377479172994185, -260.0660241030690258 ) ) ;
#87229=CARTESIAN_POINT ( 'NONE',  ( -109.6009009841024948, -280.5213961754714092, -254.2848444726273840 ) ) ;
#87230=CARTESIAN_POINT ( 'NONE',  ( 19.83368846760263438, -288.2847123798981670, -219.5919977501857261 ) ) ;
#87231=CARTESIAN_POINT ( 'NONE',  ( -111.5958314136155707, -286.6877879851134026, -259.8100689390566913 ) ) ;
#87232=CARTESIAN_POINT ( 'NONE',  ( -91.32752230076842181, -277.9608483952919755, -325.3405278219412935 ) ) ;
#87234=CARTESIAN_POINT ( 'NONE',  ( -111.3932513481078956, -270.6953707840982588, -259.2191041581176023 ) ) ;
#87236=CARTESIAN_POINT ( 'NONE',  ( 37.79695028007690638, -291.5243124805288062, -261.9116984636203824 ) ) ;
#87237=CARTESIAN_POINT ( 'NONE',  ( -73.76376950850132630, -279.4156004762390353, -202.5049346635564120 ) ) ;
#87238=CARTESIAN_POINT ( 'NONE',  ( -16.31307777119193148, -276.1871447150635390, -199.1129837178100388 ) ) ;
#87241=CARTESIAN_POINT ( 'NONE',  ( -106.6662871844225293, -293.4805209788415823, -237.0123917617630980 ) ) ;
#87242=CARTESIAN_POINT ( 'NONE',  ( -95.24082199233411927, -271.4644771141079787, -221.1306688775227656 ) ) ;
#87244=CARTESIAN_POINT ( 'NONE',  ( -108.9463045563752530, -278.2519848656275485, -255.7804320126150230 ) ) ;
#87245=CARTESIAN_POINT ( 'NONE',  ( -5.436094395339358343, -277.8467150533444965, -340.0033540384137609 ) ) ;
#87246=CARTESIAN_POINT ( 'NONE',  ( -71.95809676584293868, -299.0103631228081440, -205.4077555996138358 ) ) ;
#87247=CARTESIAN_POINT ( 'NONE',  ( -106.7978608999653147, -283.1908966454601000, -303.0515132556267872 ) ) ;
#87248=CARTESIAN_POINT ( 'NONE',  ( -75.21544796164317859, -291.3244537175978621, -333.9649458097078991 ) ) ;
#87249=CARTESIAN_POINT ( 'NONE',  ( -100.9822293102898811, -298.6313532685761061, -228.2351689511953623 ) ) ;
#87250=CARTESIAN_POINT ( 'NONE',  ( -99.60779319749049421, -298.3515458704301295, -225.7411406964684204 ) ) ;
#87251=CARTESIAN_POINT ( 'NONE',  ( 35.56725716330633702, -295.7699498231250459, -287.2792209464835764 ) ) ;
#87252=CARTESIAN_POINT ( 'NONE',  ( -33.42512046158628181, -281.0025978067237702, -345.1047820624272049 ) ) ;
#87253=CARTESIAN_POINT ( 'NONE',  ( -54.56716909451176889, -271.8498166174089761, -197.7310276724736866 ) ) ;
#87254=CARTESIAN_POINT ( 'NONE',  ( -1.365439685353753152, -288.1213139819946605, -203.1885856401416675 ) ) ;
#87255=CARTESIAN_POINT ( 'NONE',  ( 23.75956779660924667, -287.0324845419196436, -310.8915847506417549 ) ) ;
#87256=CARTESIAN_POINT ( 'NONE',  ( -111.2738350685697242, -271.9824026107303325, -296.3714058503458659 ) ) ;
#87258=CARTESIAN_POINT ( 'NONE',  ( -75.38617875257762080, -288.1239010411518962, -336.6274287234946314 ) ) ;
#87259=CARTESIAN_POINT ( 'NONE',  ( 10.12578800294857473, -288.0433894995334754, -325.9160342701869695 ) ) ;
#87261=CARTESIAN_POINT ( 'NONE',  ( -75.96299195399845416, -286.6290074716606568, -204.0437260719109815 ) ) ;
#87262=CARTESIAN_POINT ( 'NONE',  ( -61.79290780238834202, -277.7120218781069525, -339.2205844277083884 ) ) ;
#87263=EDGE_CURVE ( 'NONE', #56563, #30942, #83807, .T. ) ;
#87264=CARTESIAN_POINT ( 'NONE',  ( 6.331528368509314220, -291.5505444604578429, -207.3203246681044050 ) ) ;
#87265=CARTESIAN_POINT ( 'NONE',  ( -110.1255247843209304, -284.8904710376473304, -295.1769930403011131 ) ) ;
#87266=CARTESIAN_POINT ( 'NONE',  ( 8.117822137980358121, -282.1809137328357906, -209.0080948386793125 ) ) ;
#87267=CARTESIAN_POINT ( 'NONE',  ( -16.14358460938926143, -283.1187657124955876, -344.4189854317366439 ) ) ;
#87268=CARTESIAN_POINT ( 'NONE',  ( -22.19416355412491271, -280.5846993978017849, -198.8764832698838063 ) ) ;
#87269=CARTESIAN_POINT ( 'NONE',  ( 197.8073114025361292, 285.2187192818669246, -111.8627074968393202 ) ) ;
#87270=CARTESIAN_POINT ( 'NONE',  ( -92.29731272663953234, -279.8399450608151824, -321.2292675588906832 ) ) ;
#87271=CARTESIAN_POINT ( 'NONE',  ( 43.96814812851462051, 12.86298614219447245, -331.2283216785375544 ) ) ;
#87272=CARTESIAN_POINT ( 'NONE',  ( 137.3404605090900930, 179.3035625165208273, -238.6278596830658785 ) ) ;
#87273=CARTESIAN_POINT ( 'NONE',  ( -67.11387441388059472, -272.8487596632852501, -203.5176167432603904 ) ) ;
#87274=CARTESIAN_POINT ( 'NONE',  ( -81.84122124445936208, -295.1478143521354127, -333.1901907159369784 ) ) ;
#87275=CARTESIAN_POINT ( 'NONE',  ( -46.67462993100657087, -155.6783835708859556, -361.6360932913781312 ) ) ;
#87276=CARTESIAN_POINT ( 'NONE',  ( -105.1639677063337217, -271.6979495732385885, -234.8427339630296444 ) ) ;
#87277=CARTESIAN_POINT ( 'NONE',  ( -23.26172385449286395, -296.7307687885535756, -343.3013181649975536 ) ) ;
#87278=CARTESIAN_POINT ( 'NONE',  ( 35.45113976354100060, -289.0011581321349468, -280.5744514599383592 ) ) ;
#87280=CARTESIAN_POINT ( 'NONE',  ( -2.064903851216415287, -295.5378146961030552, -338.5400579722356156 ) ) ;
#87281=CARTESIAN_POINT ( 'NONE',  ( 19.55917037978895934, -287.3968706103750037, -224.5124927996667168 ) ) ;
#87282=CARTESIAN_POINT ( 'NONE',  ( -102.4493285647804015, -272.0048365429831847, -229.8334826128313466 ) ) ;
#87283=CARTESIAN_POINT ( 'NONE',  ( 17.45358104984482850, -295.0967238557605583, -324.3036423813090323 ) ) ;
#87284=CARTESIAN_POINT ( 'NONE',  ( 38.01158975573933674, -294.2389679511756526, -285.8984474558842521 ) ) ;
#87286=CARTESIAN_POINT ( 'NONE',  ( -96.76259796540551861, -291.3123076784474961, -227.8709322712328742 ) ) ;
#87288=CARTESIAN_POINT ( 'NONE',  ( -104.3435756380947339, -274.9327569839260264, -235.3185650403014222 ) ) ;
#87289=CARTESIAN_POINT ( 'NONE',  ( 2.226106963450188214, -273.3647149346820697, -204.7684555858694466 ) ) ;
#87291=CARTESIAN_POINT ( 'NONE',  ( -82.19789247943079147, -278.9658142037412745, -207.8515274319058221 ) ) ;
#87292=CARTESIAN_POINT ( 'NONE',  ( 21.32980628138984258, -273.3290783019095898, -225.5731929472714228 ) ) ;
#87293=CARTESIAN_POINT ( 'NONE',  ( -36.74731744702084768, -275.1394666428234927, -197.0419471297055054 ) ) ;
#87294=CARTESIAN_POINT ( 'NONE',  ( 34.60240978813735069, -276.3133755742737776, -256.6697521988016319 ) ) ;
#87295=CARTESIAN_POINT ( 'NONE',  ( -105.9381947329436571, -274.7369086618808183, -237.6732771360743470 ) ) ;
#87296=CARTESIAN_POINT ( 'NONE',  ( 35.63934254584228967, -273.8122443555967038, -289.1274233249697545 ) ) ;
#87297=CARTESIAN_POINT ( 'NONE',  ( -88.56736834861571595, -296.4450846996291489, -322.5841760501292015 ) ) ;
#87298=CARTESIAN_POINT ( 'NONE',  ( 27.67018288197493092, -292.5941174617131537, -304.9493720598764526 ) ) ;
#87300=CARTESIAN_POINT ( 'NONE',  ( -59.64117956998753556, -277.8258070894528942, -343.9971154274811624 ) ) ;
#87301=CARTESIAN_POINT ( 'NONE',  ( -21.93609811957808731, -274.4217895716409430, -199.0051971964152813 ) ) ;
#87302=CARTESIAN_POINT ( 'NONE',  ( -70.83513091964725561, -284.3043433101905748, -201.5753028104321629 ) ) ;
#87303=CARTESIAN_POINT ( 'NONE',  ( -111.9580283749157701, -298.6686313515486404, -261.2819118079733585 ) ) ;
#87305=CARTESIAN_POINT ( 'NONE',  ( -19.76718857806303120, -285.4811144340898181, -199.3418370075646635 ) ) ;
#87306=CARTESIAN_POINT ( 'NONE',  ( -103.0452667296297591, -277.2503966162068991, -236.1759650251008793 ) ) ;
#87307=CARTESIAN_POINT ( 'NONE',  ( -101.1023658560115877, -276.6259270113345110, -307.2052025868670171 ) ) ;
#87308=CARTESIAN_POINT ( 'NONE',  ( -111.6093470310158580, -286.4134885082714845, -281.1731576528224537 ) ) ;
#87309=CARTESIAN_POINT ( 'NONE',  ( 35.23197956886108528, -276.6122843233832214, -259.3134808580199433 ) ) ;
#87311=CARTESIAN_POINT ( 'NONE',  ( 29.25833729346708978, -273.4658279134842473, -233.2272293124265730 ) ) ;
#87312=CARTESIAN_POINT ( 'NONE',  ( -93.60680092389856100, -281.2440130133224443, -220.5186976893350845 ) ) ;
#87314=CARTESIAN_POINT ( 'NONE',  ( -15.84695292629675833, -288.2480831434349398, -197.8685868777397161 ) ) ;
#87316=CARTESIAN_POINT ( 'NONE',  ( 24.12504669051080342, -290.9676885813409513, -227.2984240255767361 ) ) ;
#87317=CARTESIAN_POINT ( 'NONE',  ( 82.16537594709545544, -298.2571283212178059, -196.8956743398162246 ) ) ;
#87318=CARTESIAN_POINT ( 'NONE',  ( -36.46212291700452823, -296.8583261757528362, -196.9642272592394363 ) ) ;
#87319=CARTESIAN_POINT ( 'NONE',  ( -82.46132286242755072, -289.5685795514277743, -211.3462335369621314 ) ) ;
#87320=CARTESIAN_POINT ( 'NONE',  ( -65.60899210820664962, -198.9355752380678553, -358.8784014864789924 ) ) ;
#87321=CARTESIAN_POINT ( 'NONE',  ( -73.79734911780855100, -295.5678831107678661, -204.8173440081091883 ) ) ;
#87322=CARTESIAN_POINT ( 'NONE',  ( -107.1054198436791154, -288.6324708229527687, -301.4060540099637819 ) ) ;
#87323=CARTESIAN_POINT ( 'NONE',  ( -18.51206549728809136, -284.4058086775550009, -341.7715478998489402 ) ) ;
#87324=CARTESIAN_POINT ( 'NONE',  ( -105.7568951107252104, -283.2219364173413396, -237.2954997853219936 ) ) ;
#87325=CARTESIAN_POINT ( 'NONE',  ( -23.94052758841320383, -284.3028772952277450, -342.7198319716271726 ) ) ;
#87326=CARTESIAN_POINT ( 'NONE',  ( -65.36811900831199296, -284.2309443499473218, -337.9552278606435607 ) ) ;
#87327=CARTESIAN_POINT ( 'NONE',  ( -48.59786250117770834, -291.1745405237812179, -344.9236762516080148 ) ) ;
#87328=CARTESIAN_POINT ( 'NONE',  ( 23.61349818541550150, -275.2575915701593772, -223.3268135047993326 ) ) ;
#87330=CARTESIAN_POINT ( 'NONE',  ( -41.70236007198370487, -287.1865028781521119, -345.8081623466974861 ) ) ;
#87331=CARTESIAN_POINT ( 'NONE',  ( 38.72760953650423232, -275.4018172793528834, -258.3404622175017948 ) ) ;
#87332=CARTESIAN_POINT ( 'NONE',  ( -6.053003555348501763, -296.6187749441894539, -338.1317921208016060 ) ) ;
#87333=CARTESIAN_POINT ( 'NONE',  ( 82.64890176555634582, -299.5541904835127980, -189.2068768330456123 ) ) ;
#87335=CARTESIAN_POINT ( 'NONE',  ( -56.46323529527972340, -281.9886214271139124, -341.3231526880317688 ) ) ;
#87336=CARTESIAN_POINT ( 'NONE',  ( -68.28451945632860998, -275.4574352414505825, -338.8775205843881508 ) ) ;
#87337=CARTESIAN_POINT ( 'NONE',  ( 74.93979048022610812, -297.8354839955923126, -194.1910459442052286 ) ) ;
#87338=CARTESIAN_POINT ( 'NONE',  ( 33.99090781893561086, -275.1120745045000149, -286.4039950356229838 ) ) ;
#87339=CARTESIAN_POINT ( 'NONE',  ( 25.42838062180426917, -294.5439060555598871, -231.6556734052198010 ) ) ;
#87340=CARTESIAN_POINT ( 'NONE',  ( 29.71028046796762823, -294.8883569293827236, -299.8134582218693822 ) ) ;
#87341=CARTESIAN_POINT ( 'NONE',  ( -94.92436863411488446, -286.9610598456816888, -223.8414499721200457 ) ) ;
#87342=CARTESIAN_POINT ( 'NONE',  ( 15.02106687614145741, -294.1983839140704617, -214.6400628544085976 ) ) ;
#87343=CARTESIAN_POINT ( 'NONE',  ( 33.99773281531482638, -295.2197441220977225, -298.0013708590839769 ) ) ;
#87344=CARTESIAN_POINT ( 'NONE',  ( -108.1744287244692515, -296.6190727759282595, -252.6542251949486797 ) ) ;
#87345=CARTESIAN_POINT ( 'NONE',  ( -112.3040877319867690, -292.5051888308561843, -274.0315578631796143 ) ) ;
#87346=CARTESIAN_POINT ( 'NONE',  ( -5.453581932983436076, -282.8107860758286165, -340.4478351442622852 ) ) ;
#87347=CARTESIAN_POINT ( 'NONE',  ( -95.96500942038261428, -271.3468808658288935, -222.3449104624316135 ) ) ;
#87348=CARTESIAN_POINT ( 'NONE',  ( 24.70452958863816662, -286.7797811988014587, -224.7621554673708317 ) ) ;
#87349=CARTESIAN_POINT ( 'NONE',  ( -86.16238213979377747, -279.7125912528277922, -326.8953769566107894 ) ) ;
#87351=CARTESIAN_POINT ( 'NONE',  ( -65.22995255942416293, -284.4744307031965604, -202.4146387939862279 ) ) ;
#87352=CARTESIAN_POINT ( 'NONE',  ( 24.19572886757650565, -286.1347439309681704, -313.3238464601024020 ) ) ;
#87353=CARTESIAN_POINT ( 'NONE',  ( -98.41786475236470721, -277.2971497485578425, -225.5061226893401169 ) ) ;
#87354=CARTESIAN_POINT ( 'NONE',  ( -104.9628119525177112, -256.0684274861638983, -326.9234398911233939 ) ) ;
#87355=CARTESIAN_POINT ( 'NONE',  ( -102.2902356206279819, -284.5143087649622657, -236.8995552749194928 ) ) ;
#87356=CARTESIAN_POINT ( 'NONE',  ( 21.31590875015975683, -283.4240054882389472, -319.6286898785173776 ) ) ;
#87357=CARTESIAN_POINT ( 'NONE',  ( -102.1092041658163225, -289.0680171929629410, -311.6656420689378706 ) ) ;
#87358=CARTESIAN_POINT ( 'NONE',  ( -68.66767518564732597, -279.0571418358229607, -339.8384812578836431 ) ) ;
#87359=CARTESIAN_POINT ( 'NONE',  ( -6.756365149318233065, -277.9741672813127593, -340.5025656116278014 ) ) ;
#87360=CARTESIAN_POINT ( 'NONE',  ( -107.6177356582538209, -278.6471574995300671, -250.5593167686149343 ) ) ;
#87361=CARTESIAN_POINT ( 'NONE',  ( -40.87753351654002643, -275.9874786500002415, -195.7492853401443256 ) ) ;
#87362=CARTESIAN_POINT ( 'NONE',  ( 15.43816516568050723, -292.7733411504802916, -214.2228942956865581 ) ) ;
#87363=CARTESIAN_POINT ( 'NONE',  ( -75.57965824074560146, -287.5850235820369676, -334.4831221231992231 ) ) ;
#87364=CARTESIAN_POINT ( 'NONE',  ( -6.232385340799044826, -294.0541992570694561, -200.7865678907699305 ) ) ;
#87365=CARTESIAN_POINT ( 'NONE',  ( 33.04311923035042753, -292.7430299370837474, -290.9050678882197758 ) ) ;
#87366=CARTESIAN_POINT ( 'NONE',  ( -0.7510309649830725354, -294.2188064752875789, -333.6106804635929848 ) ) ;
#87367=CARTESIAN_POINT ( 'NONE',  ( -50.52678245010447711, -292.9672198073618006, -194.8121529789007980 ) ) ;
#87368=CARTESIAN_POINT ( 'NONE',  ( 35.80492689081132340, -282.2160274776437632, -271.3068100294576084 ) ) ;
#87371=CARTESIAN_POINT ( 'NONE',  ( -40.41404922764577634, -296.9348465727555322, -193.6798768933045949 ) ) ;
#87372=CARTESIAN_POINT ( 'NONE',  ( -70.58748147724664079, -290.1304078894370946, -339.7155494786653662 ) ) ;
#87373=CARTESIAN_POINT ( 'NONE',  ( -30.35280132281144105, -281.1042205922930179, -345.8028887301368854 ) ) ;
#87374=CARTESIAN_POINT ( 'NONE',  ( 24.12788664585239573, -288.5026344928243134, -316.6993764031540195 ) ) ;
#87376=CARTESIAN_POINT ( 'NONE',  ( -42.67990905482616881, -286.3162642173693371, -197.5227308216707911 ) ) ;
#87377=DIRECTION ( 'NONE',  ( -1.000000000000000000, -0.000000000000000000, -0.000000000000000000 ) ) ;
#87378=CARTESIAN_POINT ( 'NONE',  ( 159.3374055019249909, 220.0097216543477430, -203.8079738436954642 ) ) ;
#87379=CARTESIAN_POINT ( 'NONE',  ( 198.4972914423243822, 285.9627626194107961, -96.27642562114702685 ) ) ;
#87380=CARTESIAN_POINT ( 'NONE',  ( -54.52080894794085708, -279.0230250053349437, -199.1928460675015060 ) ) ;
#87381=CARTESIAN_POINT ( 'NONE',  ( -95.85018299386948115, -278.0905842776803638, -226.1703470308495696 ) ) ;
#87382=CARTESIAN_POINT ( 'NONE',  ( -49.71165681030664985, -273.5653706364552704, -194.3288540074505590 ) ) ;
#87383=CARTESIAN_POINT ( 'NONE',  ( 27.10728642065183891, -24.65249435300752978, -342.5275202601461046 ) ) ;
#87384=CARTESIAN_POINT ( 'NONE',  ( -40.96217823716339979, -278.5821964103578239, -194.0230704717859851 ) ) ;
#87385=CARTESIAN_POINT ( 'NONE',  ( -13.01666320200853022, -280.7547668883113943, -340.9860258191369553 ) ) ;
#87386=CARTESIAN_POINT ( 'NONE',  ( -53.05748494590894637, -297.0109501695598624, -344.7586558807576580 ) ) ;
#87387=CARTESIAN_POINT ( 'NONE',  ( -28.10477759675800513, -292.6647679518334826, -197.8350368730701518 ) ) ;
#87388=CARTESIAN_POINT ( 'NONE',  ( -42.71658813141468869, -287.8060606753376192, -343.7084080248773716 ) ) ;
#87389=CARTESIAN_POINT ( 'NONE',  ( -96.86245927666115563, -273.8583029697116444, -221.6518418534377304 ) ) ;
#87390=CARTESIAN_POINT ( 'NONE',  ( -101.2155899136548527, -297.2018741531614978, -235.0181383664189525 ) ) ;
#87391=ORIENTED_EDGE ( 'NONE', *, *, #76250, .T. ) ;
#87393=CARTESIAN_POINT ( 'NONE',  ( -42.35931087744771872, -281.9094864688591997, -194.9678969269052402 ) ) ;
#87394=CARTESIAN_POINT ( 'NONE',  ( -19.47246110956689336, -281.3669857476694460, -199.2106742646069222 ) ) ;
#87395=CARTESIAN_POINT ( 'NONE',  ( -112.7576276996449565, -280.1892171748334590, -280.0725231107722948 ) ) ;
#87396=CARTESIAN_POINT ( 'NONE',  ( 35.80031659018471402, -280.6594826537344147, -274.0562279770529699 ) ) ;
#87397=CARTESIAN_POINT ( 'NONE',  ( -36.71087157183738015, -272.5400945535506594, -196.6579488219028349 ) ) ;
#87400=CARTESIAN_POINT ( 'NONE',  ( 37.47533411851565432, -276.1348917514042114, -252.7947693400713263 ) ) ;
#87401=CARTESIAN_POINT ( 'NONE',  ( 31.85812037710185862, -277.1731482225920900, -241.3067646063770724 ) ) ;
#87402=CARTESIAN_POINT ( 'NONE',  ( -94.77994920763046593, -276.4397225151909083, -320.7541119048909763 ) ) ;
#87405=CARTESIAN_POINT ( 'NONE',  ( 0.07405726863351481948, -284.5366465922003272, -335.7860257773597255 ) ) ;
#87406=CARTESIAN_POINT ( 'NONE',  ( -98.42874208005309811, -290.3075701170967591, -230.0077797776543491 ) ) ;
#87407=CARTESIAN_POINT ( 'NONE',  ( 28.61539165901615789, -286.3833291750647732, -230.7239276617104906 ) ) ;
#87408=CARTESIAN_POINT ( 'NONE',  ( -78.96475283924839061, -281.8617958153433847, -331.5615713691366864 ) ) ;
#87409=CARTESIAN_POINT ( 'NONE',  ( -74.10678701983255223, -282.1252905895308913, -334.1663762892271166 ) ) ;
#87410=CARTESIAN_POINT ( 'NONE',  ( -3.926670217352778991, -284.5762952634519820, -203.8423238163472035 ) ) ;
#87411=CARTESIAN_POINT ( 'NONE',  ( 11.55901319616538814, -281.9539609382625258, -215.6267527243214488 ) ) ;
#87412=CARTESIAN_POINT ( 'NONE',  ( 23.71396947211090733, -272.9594273849806427, -226.7822114662816944 ) ) ;
#87413=CARTESIAN_POINT ( 'NONE',  ( -95.67122081008454870, -282.2847108426046816, -319.4130120510674260 ) ) ;
#87414=CARTESIAN_POINT ( 'NONE',  ( -104.1639009116272234, -298.1007224043335100, -304.5311948212975608 ) ) ;
#87415=CARTESIAN_POINT ( 'NONE',  ( -110.1365219269036686, -279.3820639169513811, -278.8288874517366480 ) ) ;
#87416=CARTESIAN_POINT ( 'NONE',  ( -90.62187097233132249, -287.2993055969275247, -217.3398786502342261 ) ) ;
#87418=CARTESIAN_POINT ( 'NONE',  ( 38.06686676313274376, -295.5430086314377718, -275.9086037637108006 ) ) ;
#87419=CARTESIAN_POINT ( 'NONE',  ( -70.14865211115889565, -275.4841491608034403, -337.8194206447396937 ) ) ;
#87420=CARTESIAN_POINT ( 'NONE',  ( 16.56536935926178344, -287.5066981879070340, -325.1907959610214789 ) ) ;
#87421=CARTESIAN_POINT ( 'NONE',  ( 36.44089357137963958, -291.9935428719738297, -273.5435715600183357 ) ) ;
#87422=CARTESIAN_POINT ( 'NONE',  ( -64.53106175149169133, -276.0993533517874994, -338.6938779878001924 ) ) ;
#87423=CARTESIAN_POINT ( 'NONE',  ( -107.8730478718130428, -294.9958608276012910, -247.0424411260378861 ) ) ;
#87424=CARTESIAN_POINT ( 'NONE',  ( -64.26777787912008932, -293.0085004557493562, -201.9645277027552481 ) ) ;
#87425=CARTESIAN_POINT ( 'NONE',  ( -110.4683760289727132, -281.2662352645559167, -253.7030783399848985 ) ) ;
#87427=CARTESIAN_POINT ( 'NONE',  ( -50.36837877540950359, -293.6953018904815735, -345.6011029765929266 ) ) ;
#87428=CARTESIAN_POINT ( 'NONE',  ( 31.71605933782575804, -288.8070002019125582, -244.1887855995624648 ) ) ;
#87429=CARTESIAN_POINT ( 'NONE',  ( -98.37708703366595842, -289.4020300999017081, -225.0772527550459188 ) ) ;
#87430=EDGE_CURVE ( 'NONE', #81416, #92001, #49936, .T. ) ;
#87431=CARTESIAN_POINT ( 'NONE',  ( -75.00198021850144414, -290.9896388054556837, -333.5983716431630342 ) ) ;
#87433=CARTESIAN_POINT ( 'NONE',  ( -109.3360016495561240, -291.1836609239832114, -283.3773492239082543 ) ) ;
#87436=CARTESIAN_POINT ( 'NONE',  ( -69.17820966355287737, -290.6667542940334101, -340.0493156626847053 ) ) ;
#87437=CARTESIAN_POINT ( 'NONE',  ( -70.48788889747339681, -277.6374449138581326, -202.6873640045662057 ) ) ;
#87438=CARTESIAN_POINT ( 'NONE',  ( -112.6977213941364937, -279.0829151822152880, -254.5744817359279466 ) ) ;
#87439=CARTESIAN_POINT ( 'NONE',  ( 36.96571459157146933, -280.9664776829865218, -250.2075776547380599 ) ) ;
#87440=CARTESIAN_POINT ( 'NONE',  ( 25.16257708171830743, -286.1121439427332120, -311.8359330059347485 ) ) ;
#87442=CARTESIAN_POINT ( 'NONE',  ( -94.88319868027859627, -277.3446380700085001, -223.4586507975719485 ) ) ;
#87443=CARTESIAN_POINT ( 'NONE',  ( -92.93426618295407593, -281.8497423685461172, -320.7236659856005758 ) ) ;
#87445=CARTESIAN_POINT ( 'NONE',  ( -84.12643378733078237, -277.9024122162133494, -210.0124553379182544 ) ) ;
#87446=CARTESIAN_POINT ( 'NONE',  ( -106.7318251203581099, -283.0524995122739256, -303.0184764554630306 ) ) ;
#87447=CARTESIAN_POINT ( 'NONE',  ( -110.3506725206230072, -273.4267192413486782, -264.9115845521561710 ) ) ;
#87448=CARTESIAN_POINT ( 'NONE',  ( -33.38316814304199198, -299.4159035733547398, -193.8534013558464153 ) ) ;
#87449=CARTESIAN_POINT ( 'NONE',  ( -11.25044979024342773, -276.3692630959180860, -338.5618081739960417 ) ) ;
#87450=CARTESIAN_POINT ( 'NONE',  ( -5.903989809654467180, -296.6390399639862494, -338.4542235263243697 ) ) ;
#87451=CARTESIAN_POINT ( 'NONE',  ( -34.66469536096866477, -289.1860616094461420, -347.3145691722260722 ) ) ;
#87452=CARTESIAN_POINT ( 'NONE',  ( 31.07788996442805285, -280.0518135727807589, -302.5478941078378057 ) ) ;
#87453=CARTESIAN_POINT ( 'NONE',  ( -0.8019872655570401410, -292.3571057214098232, -202.5831762283037847 ) ) ;
#87454=CARTESIAN_POINT ( 'NONE',  ( -82.70135900316022060, -288.7486863419639462, -327.8581595943308002 ) ) ;
#87455=CARTESIAN_POINT ( 'NONE',  ( 34.44767913258165493, -291.8337937117538559, -292.2459588730054065 ) ) ;
#87458=CARTESIAN_POINT ( 'NONE',  ( -90.64194189747172459, -289.3406535356612039, -320.4057245494398671 ) ) ;
#87460=CARTESIAN_POINT ( 'NONE',  ( 33.63727689354109174, -288.1191482891186979, -240.9852545110913979 ) ) ;
#87461=CARTESIAN_POINT ( 'NONE',  ( -105.5937364680635966, -287.2662352645559167, -254.8156830097664738 ) ) ;
#87462=CARTESIAN_POINT ( 'NONE',  ( -13.86543179726718833, -293.8135163188520096, -343.4479501600656022 ) ) ;
#87463=CARTESIAN_POINT ( 'NONE',  ( -52.80148409090261197, -284.5613071630124296, -345.3438468166185658 ) ) ;
#87464=CARTESIAN_POINT ( 'NONE',  ( -107.3543529578805078, -284.6610613146342530, -249.5163129704913842 ) ) ;
#87465=CARTESIAN_POINT ( 'NONE',  ( 19.36877850266219880, -276.2092558774691042, -223.6153685185697100 ) ) ;
#87466=CARTESIAN_POINT ( 'NONE',  ( -28.73071693741689003, -292.9626700724140846, -344.5597412658509597 ) ) ;
#87467=CARTESIAN_POINT ( 'NONE',  ( -35.36433102320749100, -272.8724076525500664, -196.9781112787953248 ) ) ;
#87469=CARTESIAN_POINT ( 'NONE',  ( 5.045406874201050940, -57.93311274753654061, -355.0152878038887820 ) ) ;
#87470=CARTESIAN_POINT ( 'NONE',  ( -39.11160818181522103, -294.7405154851434759, -347.3196244461289552 ) ) ;
#87471=CARTESIAN_POINT ( 'NONE',  ( -7.703651408092746067, -288.3638230883290134, -202.0756856551316787 ) ) ;
#87472=CARTESIAN_POINT ( 'NONE',  ( -108.0845627511785807, -297.2520945643541950, -300.1116742640614348 ) ) ;
#87473=CARTESIAN_POINT ( 'NONE',  ( -41.33678258224720992, -286.6519756750923307, -197.3559177859472982 ) ) ;
#87474=CARTESIAN_POINT ( 'NONE',  ( -101.6874254727223246, -278.1634744556908458, -228.4027054707015623 ) ) ;
#87475=CARTESIAN_POINT ( 'NONE',  ( 29.49019281657561109, -294.6993810122234549, -308.5056728672675490 ) ) ;
#87476=CARTESIAN_POINT ( 'NONE',  ( 11.59960011635695309, -286.5208722300635031, -328.1975650402567339 ) ) ;
#87477=CARTESIAN_POINT ( 'NONE',  ( 37.44047841697738477, -294.1145115046701903, -288.6747107508439854 ) ) ;
#87478=CARTESIAN_POINT ( 'NONE',  ( -47.00146186372176516, -292.2593546115554659, -197.9817252665747276 ) ) ;
#87479=FACE_OUTER_BOUND ( 'NONE', #40850, .T. ) ;
#87481=CARTESIAN_POINT ( 'NONE',  ( 103.6749136202614778, 114.2737147221711211, -279.7089131146261138 ) ) ;
#87482=CARTESIAN_POINT ( 'NONE',  ( 30.79393473868758591, -288.6261657213288458, -236.0064529106052760 ) ) ;
#87483=CARTESIAN_POINT ( 'NONE',  ( -115.3430155898818299, -281.8380690714489560, -288.1317622949166548 ) ) ;
#87485=CARTESIAN_POINT ( 'NONE',  ( -113.6149008061959194, -278.0283247093928480, -260.1731331670051190 ) ) ;
#87486=CARTESIAN_POINT ( 'NONE',  ( 34.48735314361493920, -283.2814240054922834, -249.3702739330317968 ) ) ;
#87487=CARTESIAN_POINT ( 'NONE',  ( 7.635230013240764890, -59.72540331351240894, -353.5597951569748147 ) ) ;
#87488=CARTESIAN_POINT ( 'NONE',  ( -96.72602834267753735, -282.4768190808816257, -318.4660678217218788 ) ) ;
#87489=CARTESIAN_POINT ( 'NONE',  ( -26.28468064830018847, -286.9903124395260647, -344.0274140495475308 ) ) ;
#87490=CARTESIAN_POINT ( 'NONE',  ( -36.96997225697152345, -275.9172012707707040, -194.5843838876608913 ) ) ;
#87491=CARTESIAN_POINT ( 'NONE',  ( -77.55107103287573977, -297.9890958341909482, -209.2987225683046120 ) ) ;
#87493=CARTESIAN_POINT ( 'NONE',  ( -18.10745509621242277, -293.4837920332224144, -341.2926856711375194 ) ) ;
#87494=CARTESIAN_POINT ( 'NONE',  ( -95.83367969966693067, -279.8779490945777866, -220.4209434580480718 ) ) ;
#87495=CARTESIAN_POINT ( 'NONE',  ( -19.01694518221568941, -276.8096177405436720, -341.0237202285427429 ) ) ;
#87496=CARTESIAN_POINT ( 'NONE',  ( -74.55053736222001248, -278.8919499869463721, -207.3792141205761368 ) ) ;
#87497=CARTESIAN_POINT ( 'NONE',  ( 30.96870528085740304, -276.1810438587848466, -235.5016713180875740 ) ) ;
#87498=CARTESIAN_POINT ( 'NONE',  ( -77.66412260773562082, -276.4999882806125697, -335.6577557231277638 ) ) ;
#87500=CARTESIAN_POINT ( 'NONE',  ( -74.76067976648381830, -275.5496681823021845, -335.4179607720236618 ) ) ;
#87502=CARTESIAN_POINT ( 'NONE',  ( -105.4243873815916430, -297.5259267141387909, -305.1670114128638147 ) ) ;
#87506=CARTESIAN_POINT ( 'NONE',  ( -68.92049531987663613, -286.7065460484066648, -204.1883253691638913 ) ) ;
#87507=CARTESIAN_POINT ( 'NONE',  ( -113.3144487282843755, -286.3526147049877295, -267.1794917998780647 ) ) ;
#87508=CARTESIAN_POINT ( 'NONE',  ( 0.2281604315425367902, -285.9149977900521549, -207.5932631964456050 ) ) ;
#87509=CARTESIAN_POINT ( 'NONE',  ( -110.0779924788421198, -276.7881326928743420, -282.9208106700475582 ) ) ;
#87510=CARTESIAN_POINT ( 'NONE',  ( -97.59095512839444098, -287.0091669695266319, -226.9701629338598252 ) ) ;
#87511=CARTESIAN_POINT ( 'NONE',  ( -74.84208895854072807, -278.0233813588476437, -206.8640880892528742 ) ) ;
#87512=CARTESIAN_POINT ( 'NONE',  ( -76.50940247791791649, -278.6689211493159064, -332.3894928956623289 ) ) ;
#87514=CARTESIAN_POINT ( 'NONE',  ( 33.30329851965409915, -276.2903645851201873, -288.9963697350226539 ) ) ;
#87516=CARTESIAN_POINT ( 'NONE',  ( 38.51009246984892798, -282.5098452898087658, -282.7179164840283079 ) ) ;
#87517=CARTESIAN_POINT ( 'NONE',  ( -44.40731385203950765, -283.6314734543273630, -347.0277734786789665 ) ) ;
#87521=CARTESIAN_POINT ( 'NONE',  ( 13.78789841822058904, -290.2052667678747184, -326.3434982694111000 ) ) ;
#87523=CARTESIAN_POINT ( 'NONE',  ( -96.02365161109059954, -288.5719215777939439, -319.4704125664965204 ) ) ;
#87524=CARTESIAN_POINT ( 'NONE',  ( -65.62572121608263842, -296.8696999052388037, -202.8880427721977924 ) ) ;
#87525=CARTESIAN_POINT ( 'NONE',  ( -4.639949800427709548, -291.8203395988667808, -200.7629261049724505 ) ) ;
#87526=CARTESIAN_POINT ( 'NONE',  ( 24.81282923063587020, -286.5743261034620559, -309.9530645397802004 ) ) ;
#87527=CARTESIAN_POINT ( 'NONE',  ( 31.34076396985507884, -288.4120111772829205, -244.3362754279621640 ) ) ;
#87528=CARTESIAN_POINT ( 'NONE',  ( -54.42813229853333468, -297.7662352645559167, -345.3683826091709648 ) ) ;
#87529=CARTESIAN_POINT ( 'NONE',  ( -71.10632659307661640, -287.4966203649944987, -337.5174909502709966 ) ) ;
#87530=CARTESIAN_POINT ( 'NONE',  ( -80.75601236308186515, -284.5985298707938114, -329.4039128301236588 ) ) ;
#87531=CARTESIAN_POINT ( 'NONE',  ( -76.24279594863611464, -293.5340424947768270, -205.9836385051075922 ) ) ;
#87534=CARTESIAN_POINT ( 'NONE',  ( -34.14802657023491150, -300.0119829776966185, -194.8000747783010524 ) ) ;
#87536=CARTESIAN_POINT ( 'NONE',  ( 19.47097385672049796, -281.4003305579699372, -316.4777359957691942 ) ) ;
#87537=CARTESIAN_POINT ( 'NONE',  ( -99.19585473824058397, -281.9762871659203824, -312.8670508382804201 ) ) ;
#87538=CARTESIAN_POINT ( 'NONE',  ( 37.91037156935676933, -292.9439976829007719, -285.8944539526964945 ) ) ;
#87539=CARTESIAN_POINT ( 'NONE',  ( -108.1596390510478187, -271.0750294385023835, -248.6730993082246925 ) ) ;
#87540=CARTESIAN_POINT ( 'NONE',  ( 36.12435790985168182, -273.7912828932889511, -282.6741484721150641 ) ) ;
#87541=CARTESIAN_POINT ( 'NONE',  ( -60.68832360411418847, -299.0581455123403316, -200.6209957712173377 ) ) ;
#87543=CARTESIAN_POINT ( 'NONE',  ( -81.30394289193519342, -293.8802244051389607, -332.4035795776117084 ) ) ;
#87544=CARTESIAN_POINT ( 'NONE',  ( -2.851656814702925313, -296.0120871980672064, -335.3673625330421828 ) ) ;
#87546=CARTESIAN_POINT ( 'NONE',  ( -38.33425059091678833, -295.8677434835836380, -343.5158619919911871 ) ) ;
#87548=CARTESIAN_POINT ( 'NONE',  ( -109.9143609314994023, -282.3124927603950027, -290.6494325634084817 ) ) ;
#87549=CARTESIAN_POINT ( 'NONE',  ( -90.04586497955105528, -297.2817562745242981, -219.7786690494482684 ) ) ;
#87550=CARTESIAN_POINT ( 'NONE',  ( -110.6855457350264089, -284.2568996930114054, -293.8498614111003917 ) ) ;
#87551=CARTESIAN_POINT ( 'NONE',  ( 35.80408693258499397, -283.7139639184255202, -289.3086253683503628 ) ) ;
#87552=CARTESIAN_POINT ( 'NONE',  ( 39.58297291944533214, -287.2697232695270486, -274.4260518540313001 ) ) ;
#87553=CARTESIAN_POINT ( 'NONE',  ( -33.38669500999364459, -290.1018730315056473, -195.6195603438067110 ) ) ;
#87555=CARTESIAN_POINT ( 'NONE',  ( -22.58714906154741442, -279.4334352304951494, -194.8983413833674376 ) ) ;
#87557=CARTESIAN_POINT ( 'NONE',  ( 39.58706461736020543, -279.0523547857347353, -270.3937649182068981 ) ) ;
#87559=CARTESIAN_POINT ( 'NONE',  ( 29.78200958327513703, -286.7459899928995242, -300.1778632230015660 ) ) ;
#87560=CARTESIAN_POINT ( 'NONE',  ( -59.94932255653006337, -288.2587668073750820, -343.6440485817265653 ) ) ;
#87562=CARTESIAN_POINT ( 'NONE',  ( -110.8947425426318318, -298.0657688213805159, -276.9915744421043087 ) ) ;
#87563=CARTESIAN_POINT ( 'NONE',  ( -97.45403635994424008, -279.3419342140627464, -317.5322249034054494 ) ) ;
#87564=CARTESIAN_POINT ( 'NONE',  ( -70.11579738028902398, -293.5018121659139752, -338.2300571174537254 ) ) ;
#87565=CARTESIAN_POINT ( 'NONE',  ( 20.53528754459697225, -280.5922171555554314, -225.8172970462405829 ) ) ;
#87566=CARTESIAN_POINT ( 'NONE',  ( 24.03026120878803695, -294.3383627706788843, -316.8636164766572847 ) ) ;
#87567=CARTESIAN_POINT ( 'NONE',  ( -5.360778727914657260, -284.5495124266410585, -201.9028469816150562 ) ) ;
#87568=CARTESIAN_POINT ( 'NONE',  ( -112.3833687534820172, -280.5363918678977484, -271.6014193245699744 ) ) ;
#87570=CARTESIAN_POINT ( 'NONE',  ( -66.15671935062889020, -294.4975776610245930, -337.6894412632343005 ) ) ;
#87573=CARTESIAN_POINT ( 'NONE',  ( 26.53095494188747239, -283.0108534428742360, -231.6328984051195050 ) ) ;
#87574=CARTESIAN_POINT ( 'NONE',  ( -109.8663645048646345, -295.9379310576269972, -279.6074175544224545 ) ) ;
#87576=CARTESIAN_POINT ( 'NONE',  ( 39.58706461736021254, -279.0523547857347921, -270.3937649182068981 ) ) ;
#87577=CARTESIAN_POINT ( 'NONE',  ( -55.28597065623892348, -273.0241447500357594, -195.6472506271032046 ) ) ;
#87578=CARTESIAN_POINT ( 'NONE',  ( -85.92744527199947413, -291.1901943325169100, -215.8098238759642982 ) ) ;
#87579=CARTESIAN_POINT ( 'NONE',  ( -102.7803826199349970, -280.5301319594593679, -236.3606751181626464 ) ) ;
#87580=CARTESIAN_POINT ( 'NONE',  ( -6.209839808988696142, -276.0683258064257757, -203.4488792625690223 ) ) ;
#87581=CARTESIAN_POINT ( 'NONE',  ( 13.16593101578489033, -283.9605066859061253, -327.4876547216936729 ) ) ;
#87582=CARTESIAN_POINT ( 'NONE',  ( 29.67075810574870331, -280.7495660452669881, -300.4268066405655304 ) ) ;
#87583=CARTESIAN_POINT ( 'NONE',  ( -36.41663272233579107, -279.0407500617605479, -345.3682255897130631 ) ) ;
#87585=CARTESIAN_POINT ( 'NONE',  ( -2.555644637146083475, -274.3326974178143587, -201.6519440078532455 ) ) ;
#87586=CARTESIAN_POINT ( 'NONE',  ( -6.699395299630709566, -294.3777681672877407, -202.5203974996412342 ) ) ;
#87589=CARTESIAN_POINT ( 'NONE',  ( 36.85605935456775484, -291.8865854144556238, -285.6907615350536958 ) ) ;
#87590=CARTESIAN_POINT ( 'NONE',  ( -74.29910333014065316, -273.0545169139391533, -207.2776089167914506 ) ) ;
#87592=CARTESIAN_POINT ( 'NONE',  ( -30.77639269453639415, -293.6536957653947297, -194.2851246914145236 ) ) ;
#87593=CARTESIAN_POINT ( 'NONE',  ( -4.771743288812468897, -279.1233781216988064, -337.9199732462171255 ) ) ;
#87594=CARTESIAN_POINT ( 'NONE',  ( -74.49979213554404112, -292.7742028081192984, -203.3739183294904649 ) ) ;
#87595=CARTESIAN_POINT ( 'NONE',  ( -20.69740580411836461, -290.8381335221212112, -343.3199823501925607 ) ) ;
#87596=CARTESIAN_POINT ( 'NONE',  ( -24.02783698658281608, -274.8816854538034704, -344.0533143627347954 ) ) ;
#87597=CARTESIAN_POINT ( 'NONE',  ( -9.426098482943086054, -278.6046351802551158, -339.3824413155019215 ) ) ;
#87598=CARTESIAN_POINT ( 'NONE',  ( 25.63266268321738650, -292.1708600324493545, -310.1510163022412598 ) ) ;
#87599=CARTESIAN_POINT ( 'NONE',  ( -6.751163037297327030, -282.3098324955339535, -201.0323995500967555 ) ) ;
#87601=CARTESIAN_POINT ( 'NONE',  ( -91.68361916541283563, -283.5208182553025722, -319.1553718120687222 ) ) ;
#87602=CARTESIAN_POINT ( 'NONE',  ( -97.46317221718877022, -280.2714837524911218, -222.7491330918078631 ) ) ;
#87603=CARTESIAN_POINT ( 'NONE',  ( 11.22892348023847120, -281.1916719194254597, -329.6657441995660065 ) ) ;
#87604=CARTESIAN_POINT ( 'NONE',  ( 12.56077744296938192, -277.3173491543691966, -328.6926098594030918 ) ) ;
#87606=CARTESIAN_POINT ( 'NONE',  ( 38.86070081911479690, -277.0104812500239291, -265.4647988023256744 ) ) ;
#87607=CARTESIAN_POINT ( 'NONE',  ( 17.36665895637874613, -289.4090924074130839, -226.6919474004047572 ) ) ;
#87610=CARTESIAN_POINT ( 'NONE',  ( -53.07894532440435853, -299.8507008661060809, -196.9774608745953799 ) ) ;
#87611=CARTESIAN_POINT ( 'NONE',  ( -95.75560999814437935, -275.9302629771005400, -316.8537058867900100 ) ) ;
#87612=CARTESIAN_POINT ( 'NONE',  ( -55.96245056272222484, -293.5758457683152187, -196.6370734048880422 ) ) ;
#87613=CARTESIAN_POINT ( 'NONE',  ( -25.38425869722593831, -291.5570391642943378, -198.1922159257624116 ) ) ;
#87614=CARTESIAN_POINT ( 'NONE',  ( -8.262206471111200656, -288.1891069550692919, -341.6067554536527382 ) ) ;
#87616=CARTESIAN_POINT ( 'NONE',  ( 36.85418429646944816, -291.8966452661995277, -252.0970267261715207 ) ) ;
#87617=CARTESIAN_POINT ( 'NONE',  ( -69.37464076112472355, -281.8807275088116739, -336.8606453119332969 ) ) ;
#87618=CARTESIAN_POINT ( 'NONE',  ( -110.3902244750873223, -292.2410733930450419, -283.5815027249457785 ) ) ;
#87619=CARTESIAN_POINT ( 'NONE',  ( -109.6050828115442499, -283.2208122014051810, -255.9142748241255561 ) ) ;
#87620=CARTESIAN_POINT ( 'NONE',  ( 30.79798100044280318, -283.2335899928863796, -297.8970460153339559 ) ) ;
#87622=CARTESIAN_POINT ( 'NONE',  ( -9.637034140845045727, -289.6401255389210405, -341.9521208772692376 ) ) ;
#87623=CARTESIAN_POINT ( 'NONE',  ( 11.34216485102379757, -281.2413471421197073, -215.8829596785950287 ) ) ;
#87624=CARTESIAN_POINT ( 'NONE',  ( -0.9787474148457222523, -291.3188778073098888, -202.9389822313664808 ) ) ;
#87625=CARTESIAN_POINT ( 'NONE',  ( 26.21803381920792475, -287.7842217834903522, -227.1598572191831238 ) ) ;
#87627=CARTESIAN_POINT ( 'NONE',  ( 28.85399186004476135, -288.5557832374823874, -309.5740911588089261 ) ) ;
#87628=CARTESIAN_POINT ( 'NONE',  ( -9.495354637964695144, -286.5931257222802628, -202.8673832001296091 ) ) ;
#87631=CARTESIAN_POINT ( 'NONE',  ( 28.51295730169438869, -295.9081890810738287, -307.9300671776576337 ) ) ;
#87632=CARTESIAN_POINT ( 'NONE',  ( -47.58224614309366984, -293.8645745941540213, -346.1795160742690882 ) ) ;
#87633=CARTESIAN_POINT ( 'NONE',  ( -109.5200206750281069, -277.4469026621178500, -282.8328312550918895 ) ) ;
#87634=CARTESIAN_POINT ( 'NONE',  ( -91.55777619641089871, -296.6528586230794531, -215.8273680456153727 ) ) ;
#87636=CARTESIAN_POINT ( 'NONE',  ( 4.916922602897884964, -291.1142213549914572, -209.9254083739679686 ) ) ;
#87637=CARTESIAN_POINT ( 'NONE',  ( -102.3681490373165985, -294.3161472493381439, -305.7098796792338362 ) ) ;
#87638=CARTESIAN_POINT ( 'NONE',  ( 20.01361989501665661, -295.4008420965192840, -316.1796064249823530 ) ) ;
#87639=CARTESIAN_POINT ( 'NONE',  ( 34.37282683833672792, -294.8323773731113420, -285.6283781040641543 ) ) ;
#87641=CARTESIAN_POINT ( 'NONE',  ( 12.16865261693645550, -292.3655376346080743, -326.9876309818918685 ) ) ;
#87643=CARTESIAN_POINT ( 'NONE',  ( -108.4779915619095192, -298.2432961741336044, -294.2840549399437577 ) ) ;
#87644=CARTESIAN_POINT ( 'NONE',  ( -109.6495107990008933, -291.3395972305177679, -282.0583913210004994 ) ) ;
#87645=CARTESIAN_POINT ( 'NONE',  ( -50.47084430307474889, -295.5577315974794033, -342.1922606709545107 ) ) ;
#87646=CARTESIAN_POINT ( 'NONE',  ( -86.01318886397322672, -279.7022791178366674, -327.9575643388695312 ) ) ;
#87647=CARTESIAN_POINT ( 'NONE',  ( -73.51758170409270576, -278.2672920774273848, -202.9325873657557224 ) ) ;
#87648=CARTESIAN_POINT ( 'NONE',  ( -3.862976237089331910, -273.8308176644274567, -201.1188311114435123 ) ) ;
#87649=CARTESIAN_POINT ( 'NONE',  ( 37.14338441879935715, -279.6448739711028111, -271.3569532551027237 ) ) ;
#87650=CARTESIAN_POINT ( 'NONE',  ( -101.2094472046138520, -277.5047043023939750, -228.7042607584561722 ) ) ;
#87651=CARTESIAN_POINT ( 'NONE',  ( -45.05918793247583665, -277.9546122624539635, -195.5399520672403639 ) ) ;
#87652=CARTESIAN_POINT ( 'NONE',  ( -92.20193278392555669, -295.9316335854428530, -221.4571472679120632 ) ) ;
#87653=CARTESIAN_POINT ( 'NONE',  ( 23.02374208698441649, -276.9449014607387198, -225.8313406892640955 ) ) ;
#87655=CARTESIAN_POINT ( 'NONE',  ( -73.85926192655631439, -289.5897492496762879, -204.4454560773035894 ) ) ;
#87656=CARTESIAN_POINT ( 'NONE',  ( -41.76055760479342638, -289.1063468511020460, -347.2474414363900337 ) ) ;
#87657=CARTESIAN_POINT ( 'NONE',  ( 8.374651001252306770, -276.6764850633429091, -210.6950165269120134 ) ) ;
#87658=CARTESIAN_POINT ( 'NONE',  ( -37.11921302921708588, -296.0547944567841796, -195.5249315462412483 ) ) ;
#87660=CARTESIAN_POINT ( 'NONE',  ( -49.30947078709969844, -285.1006280993699420, -194.4066966165096915 ) ) ;
#87663=CARTESIAN_POINT ( 'NONE',  ( -71.23061273360882240, -281.4993107491206956, -337.2821291566444302 ) ) ;
#87665=CARTESIAN_POINT ( 'NONE',  ( 35.69205627309717244, -292.2449138296782962, -262.5749610052877188 ) ) ;
#87666=CARTESIAN_POINT ( 'NONE',  ( -82.20657095559761274, -283.5722075174023757, -211.2171508925511603 ) ) ;
#87669=CARTESIAN_POINT ( 'NONE',  ( 36.81157819309344603, -291.7006130131134114, -281.9361465053453912 ) ) ;
#87670=CARTESIAN_POINT ( 'NONE',  ( -106.0047429214089476, -279.7944202747025884, -297.4134185876326342 ) ) ;
#87671=CARTESIAN_POINT ( 'NONE',  ( -16.23642890538016559, -283.9904199334760619, -344.0542662701463996 ) ) ;
#87672=CARTESIAN_POINT ( 'NONE',  ( -29.95486989272370337, -272.2248079214666063, -195.1630532701500442 ) ) ;
#87673=CARTESIAN_POINT ( 'NONE',  ( -94.95705715023834159, -285.1839775431552653, -225.5137010795961032 ) ) ;
#87674=CARTESIAN_POINT ( 'NONE',  ( 29.61468970115871713, -276.5675960214273914, -239.7056895592586159 ) ) ;
#87675=CARTESIAN_POINT ( 'NONE',  ( -18.96653808151215159, -277.6123211135574707, -341.1774659977460828 ) ) ;
#87676=CARTESIAN_POINT ( 'NONE',  ( -101.2014608117364247, -286.0245128539817188, -309.6921694911256964 ) ) ;
#87679=CARTESIAN_POINT ( 'NONE',  ( -72.07593502769803706, -295.3321009502789707, -339.0818057735624507 ) ) ;
#87680=CARTESIAN_POINT ( 'NONE',  ( 24.89174481380062431, -288.9716605667255749, -229.0505342790021643 ) ) ;
#87682=CARTESIAN_POINT ( 'NONE',  ( 25.22466315766300227, -278.6948066931273047, -320.2154176792147382 ) ) ;
#87683=CARTESIAN_POINT ( 'NONE',  ( -94.72134569164256845, -278.1646786285700728, -219.4782251284936478 ) ) ;
#87684=CARTESIAN_POINT ( 'NONE',  ( -4.925770865371022822, -290.8717779850562692, -201.3999118701938187 ) ) ;
#87685=CARTESIAN_POINT ( 'NONE',  ( -30.48587862925580083, -287.6604026744830094, -196.9360993798321431 ) ) ;
#87686=CARTESIAN_POINT ( 'NONE',  ( -86.16927336917946434, -281.1239701408817950, -214.7388013948472576 ) ) ;
#87687=CARTESIAN_POINT ( 'NONE',  ( -2.056557930385312982, -290.0194516900936605, -338.1369620161691500 ) ) ;
#87688=CARTESIAN_POINT ( 'NONE',  ( 37.68755262768855374, -283.5285420699671022, -268.5094602435746083 ) ) ;
#87689=CARTESIAN_POINT ( 'NONE',  ( -65.09309052314583255, -277.5714437409737911, -342.2426101730581536 ) ) ;
#87690=CARTESIAN_POINT ( 'NONE',  ( -35.06023292077971831, -296.1009576339022260, -195.7170838746797585 ) ) ;
#87691=CARTESIAN_POINT ( 'NONE',  ( -33.91314828073721088, -279.9274891428796082, -193.4374867841462162 ) ) ;
#87692=CARTESIAN_POINT ( 'NONE',  ( 10.05277193782247380, -300.5700594497022848, -195.9054571269808775 ) ) ;
#87695=CARTESIAN_POINT ( 'NONE',  ( -54.42813229853333468, -291.7662352645558599, -345.3683826091709648 ) ) ;
#87697=CARTESIAN_POINT ( 'NONE',  ( -97.00332737469258859, -271.4298440896898796, -223.3030235470189666 ) ) ;
#87699=CARTESIAN_POINT ( 'NONE',  ( -49.14568172656405665, -279.4053045768581569, -198.2594227186683327 ) ) ;
#87700=CARTESIAN_POINT ( 'NONE',  ( 30.88962546190047931, -276.3064280074575549, -235.5402201521648351 ) ) ;
#87702=CARTESIAN_POINT ( 'NONE',  ( -96.09797787083066112, -282.9434806833758103, -319.7830803612201294 ) ) ;
#87703=CARTESIAN_POINT ( 'NONE',  ( 12.85935342445114138, -290.1005334165959653, -324.8167002319706853 ) ) ;
#87704=CARTESIAN_POINT ( 'NONE',  ( -89.15188416617448297, -298.8595847898933471, -214.2679860340728908 ) ) ;
#87705=CARTESIAN_POINT ( 'NONE',  ( -73.10895954997174329, -298.7942267989574248, -202.5625366539127015 ) ) ;
#87706=CARTESIAN_POINT ( 'NONE',  ( 34.89289578589387730, -295.8047943557069175, -289.9596233341212042 ) ) ;
#87708=CARTESIAN_POINT ( 'NONE',  ( 28.07348933608626496, -279.0672813068800906, -234.0171857338120844 ) ) ;
#87709=CARTESIAN_POINT ( 'NONE',  ( -21.56228543215167903, -272.2755627941558032, -197.4032063387302287 ) ) ;
#87710=CARTESIAN_POINT ( 'NONE',  ( -35.19144490035210993, -287.6788166996584550, -194.1784527693881444 ) ) ;
#87711=CARTESIAN_POINT ( 'NONE',  ( -78.35870518029398113, -288.5384435926697506, -331.1826799100534231 ) ) ;
#87712=CARTESIAN_POINT ( 'NONE',  ( 204.8861976254080730, 294.6280088066694702, -54.00000000002151523 ) ) ;
#87714=CARTESIAN_POINT ( 'NONE',  ( 9.849675925451636616, -286.9917841445231943, -330.5248428514432817 ) ) ;
#87715=CARTESIAN_POINT ( 'NONE',  ( 20.37156175138847303, -287.8489544262758955, -315.1168829400816662 ) ) ;
#87717=CARTESIAN_POINT ( 'NONE',  ( -105.1651740154182306, -286.0971535812261095, -234.4497636982327435 ) ) ;
#87718=CARTESIAN_POINT ( 'NONE',  ( -13.77456064013578718, -277.0711167469324323, -339.5277835418974632 ) ) ;
#87719=CARTESIAN_POINT ( 'NONE',  ( 33.12707991427834031, -292.8609785640342125, -300.7547782340529920 ) ) ;
#87720=CARTESIAN_POINT ( 'NONE',  ( 27.76062937459834501, -281.6658322095683502, -229.3345862278431468 ) ) ;
#87721=CARTESIAN_POINT ( 'NONE',  ( 36.99760797571403970, -282.8543526781491551, -253.0882274791171369 ) ) ;
#87722=CARTESIAN_POINT ( 'NONE',  ( -18.91934070798767564, -283.1546766290548476, -345.1580238620608156 ) ) ;
#87723=CARTESIAN_POINT ( 'NONE',  ( 19.68986935376914715, -281.2413681749819716, -224.7597192176230863 ) ) ;
#87724=CARTESIAN_POINT ( 'NONE',  ( -106.6379572354042296, -276.4809262143061233, -236.9535640164627353 ) ) ;
#87725=CARTESIAN_POINT ( 'NONE',  ( -83.79983398228941383, -219.7295597296427729, -352.6263433563659078 ) ) ;
#87726=CARTESIAN_POINT ( 'NONE',  ( -79.64798785157238115, -279.6250536609471737, -332.1510719737299269 ) ) ;
#87727=CARTESIAN_POINT ( 'NONE',  ( -64.64839057758955221, -182.1492425233583390, -361.6151995916652595 ) ) ;
#87728=CARTESIAN_POINT ( 'NONE',  ( 187.6320441055845265, 269.2822349766076968, -137.7557671003276596 ) ) ;
#87729=CARTESIAN_POINT ( 'NONE',  ( -77.56114516728148089, -296.8455196481110647, -209.2569580648613226 ) ) ;
#87730=CARTESIAN_POINT ( 'NONE',  ( 39.59470444098784014, -293.0233091165462156, -267.4451949993101607 ) ) ;
#87731=CARTESIAN_POINT ( 'NONE',  ( -20.90964142997582087, -109.3750234531322434, -359.1970471300297731 ) ) ;
#87732=CARTESIAN_POINT ( 'NONE',  ( -84.83588423967957226, -295.9863936537509517, -210.5037143732127731 ) ) ;
#87733=CARTESIAN_POINT ( 'NONE',  ( -98.01813882430053582, -288.3728288070954022, -312.3929722805241340 ) ) ;
#87734=CARTESIAN_POINT ( 'NONE',  ( -63.99064704868445830, -297.2637255795025908, -339.7026515647153246 ) ) ;
#87735=CARTESIAN_POINT ( 'NONE',  ( -10.52867414003060631, -290.0101937330874193, -338.8430767880722669 ) ) ;
#87737=CARTESIAN_POINT ( 'NONE',  ( -68.12080236320932158, -296.3878132635525162, -340.6851329357700138 ) ) ;
#87738=CARTESIAN_POINT ( 'NONE',  ( -42.68488116543220912, -286.4753045616939175, -197.4825853240655249 ) ) ;
#87739=CARTESIAN_POINT ( 'NONE',  ( -37.23863709957562662, -296.8483480566467279, -193.7574484753887702 ) ) ;
#87740=CARTESIAN_POINT ( 'NONE',  ( -73.36707471665447144, -292.3895830916884506, -202.4762905216695117 ) ) ;
#87741=CARTESIAN_POINT ( 'NONE',  ( 39.44119486658600238, -294.1154316632586188, -276.0283630418419989 ) ) ;
#87742=CARTESIAN_POINT ( 'NONE',  ( -41.59495959226429562, -292.1639144248005096, -197.4352824795317645 ) ) ;
#87744=CARTESIAN_POINT ( 'NONE',  ( -110.4317800807580454, -274.7190581390205466, -250.9993558362557167 ) ) ;
#87745=CARTESIAN_POINT ( 'NONE',  ( 23.32781192550636007, -273.7194835547869616, -223.5720484397543260 ) ) ;
#87747=CARTESIAN_POINT ( 'NONE',  ( -14.61386100977054880, -276.2730603983901574, -343.9218104195533670 ) ) ;
#87748=CARTESIAN_POINT ( 'NONE',  ( -111.1409416881142960, -270.9882135121230249, -267.5870818430676081 ) ) ;
#87749=CARTESIAN_POINT ( 'NONE',  ( 27.84016578767272421, -274.1699115899199342, -305.9958289008915244 ) ) ;
#87750=CARTESIAN_POINT ( 'NONE',  ( -69.63948234451837038, -274.6962687544138930, -204.5501816681222067 ) ) ;
#87751=CARTESIAN_POINT ( 'NONE',  ( -96.47844273691961803, -274.0973830620596914, -227.0766828920960165 ) ) ;
#87752=CARTESIAN_POINT ( 'NONE',  ( -113.1714757354526029, -274.3837324972880083, -264.7240405394982190 ) ) ;
#87753=CARTESIAN_POINT ( 'NONE',  ( 23.03436878347866212, -274.1852251613643148, -315.4514396538984329 ) ) ;
#87754=CARTESIAN_POINT ( 'NONE',  ( -68.55333468295162902, -296.1248304046246744, -336.4787749857893004 ) ) ;
#87755=CARTESIAN_POINT ( 'NONE',  ( 32.08999944322635400, -292.4505204592193195, -294.8982949945201426 ) ) ;
#87756=DIRECTION ( 'NONE',  ( 0.000000000000000000, -1.000000000000000000, 0.000000000000000000 ) ) ;
#87757=CARTESIAN_POINT ( 'NONE',  ( 14.84604505116894124, -276.8326866572894573, -326.9665113025326377 ) ) ;
#87758=CARTESIAN_POINT ( 'NONE',  ( 5.175022792764202073, -274.8116094583524500, -210.9578614270271260 ) ) ;
#87759=CARTESIAN_POINT ( 'NONE',  ( -113.3278864882182972, -283.3491378818575299, -261.4505762110455862 ) ) ;
#87760=CARTESIAN_POINT ( 'NONE',  ( -109.8602776456810943, -298.8082655518210800, -250.3926887040111637 ) ) ;
#87762=CARTESIAN_POINT ( 'NONE',  ( -57.42892732028073510, -284.9834640621994595, -199.9585149068916792 ) ) ;
#87763=EDGE_CURVE ( 'NONE', #36646, #17445, #86932, .T. ) ;
#87764=CARTESIAN_POINT ( 'NONE',  ( -109.1607529504536700, -276.5585648801060756, -288.3019083407866106 ) ) ;
#87765=CARTESIAN_POINT ( 'NONE',  ( -96.57802182668140745, -276.5196006078688811, -314.0449661716374976 ) ) ;
#87767=CARTESIAN_POINT ( 'NONE',  ( -14.72095575521275634, -284.7593253708719203, -341.9223017075121902 ) ) ;
#87768=CARTESIAN_POINT ( 'NONE',  ( -5.147665521381033393, -275.6907077862326219, -204.3875763608342879 ) ) ;
#87770=CARTESIAN_POINT ( 'NONE',  ( 26.96265883984539258, -274.4946107954796162, -311.3417942069518176 ) ) ;
#87772=CARTESIAN_POINT ( 'NONE',  ( -36.79216438632334985, -282.0592019842418949, -195.1837213708406580 ) ) ;
#87774=DIRECTION ( 'NONE',  ( 0.000000000000000000, 0.000000000000000000, -1.000000000000000000 ) ) ;
#87775=CARTESIAN_POINT ( 'NONE',  ( 25.15236128287760664, -288.9013629590166943, -227.8667723274509456 ) ) ;
#87777=CARTESIAN_POINT ( 'NONE',  ( -110.9992461515954432, -288.7342405490479109, -256.1672670994903456 ) ) ;
#87779=CARTESIAN_POINT ( 'NONE',  ( -98.24251575579194196, -271.8060356762467222, -229.1323689943044997 ) ) ;
#87780=CARTESIAN_POINT ( 'NONE',  ( -110.4898117228061949, -288.8597326408641379, -257.4103788922319040 ) ) ;
#87781=CARTESIAN_POINT ( 'NONE',  ( -30.04969936926732288, -125.9919632799748683, -361.3284013991797110 ) ) ;
#87783=CARTESIAN_POINT ( 'NONE',  ( 35.71593305586371514, -286.3115636853480055, -292.4357594100327447 ) ) ;
#87784=CARTESIAN_POINT ( 'NONE',  ( -36.16051173489322679, -284.6372286024638356, -344.1516675898475910 ) ) ;
#87785=CARTESIAN_POINT ( 'NONE',  ( -109.7271653665450089, -282.4970424126898934, -293.5193965673146863 ) ) ;
#87786=CARTESIAN_POINT ( 'NONE',  ( 33.29512897756002587, -282.7066286504908135, -249.7258740607108223 ) ) ;
#87787=CARTESIAN_POINT ( 'NONE',  ( -16.07582197716827110, -283.5728422136733684, -340.3637190274759519 ) ) ;
#87788=CARTESIAN_POINT ( 'NONE',  ( -43.03238562738368955, -291.1035554964944936, -345.5011399529491882 ) ) ;
#87790=CARTESIAN_POINT ( 'NONE',  ( -71.39726666672559929, -273.9479541658585617, -201.3251659040370782 ) ) ;
#87791=CARTESIAN_POINT ( 'NONE',  ( 27.65242258729247737, -286.1436706010331363, -308.8978304606699226 ) ) ;
#87792=CARTESIAN_POINT ( 'NONE',  ( 7.234989325463415888, -274.6407946568432408, -207.5109817883472090 ) ) ;
#87793=CARTESIAN_POINT ( 'NONE',  ( 0.08817779316672660905, -296.5316065945155515, -335.0022472712446984 ) ) ;
#87795=CARTESIAN_POINT ( 'NONE',  ( -114.2704648735229114, -299.0519495502701943, -270.3937649182068981 ) ) ;
#87796=CARTESIAN_POINT ( 'NONE',  ( -61.71395680402517314, -282.0602883975840882, -339.7489571766276413 ) ) ;
#87797=CARTESIAN_POINT ( 'NONE',  ( -110.3994766756951265, -276.3247971815480923, -288.0953096142770278 ) ) ;
#87798=CARTESIAN_POINT ( 'NONE',  ( 97.44483485902340192, -298.1127538979946507, -194.1970331066050619 ) ) ;
#87799=CARTESIAN_POINT ( 'NONE',  ( 32.96034237152142765, -274.6340168712055174, -250.1423167060101775 ) ) ;
#87800=CARTESIAN_POINT ( 'NONE',  ( 30.48638752210645109, -294.6875438753584149, -241.4199154866854826 ) ) ;
#87801=CARTESIAN_POINT ( 'NONE',  ( -4.739066623368627162, -293.4336835495118976, -204.7691291320868459 ) ) ;
#87802=CARTESIAN_POINT ( 'NONE',  ( -105.5398861930802923, -286.6945283810787828, -241.4720055665673328 ) ) ;
#87803=CARTESIAN_POINT ( 'NONE',  ( 24.32808310391603257, -294.3737885216199857, -225.2452213375096903 ) ) ;
#87804=CARTESIAN_POINT ( 'NONE',  ( 35.02545210688794697, -295.1840497100538414, -295.3488295946599465 ) ) ;
#87805=CARTESIAN_POINT ( 'NONE',  ( -107.9701166240041914, -296.1412091993184390, -288.8666236863512609 ) ) ;
#87806=CARTESIAN_POINT ( 'NONE',  ( -53.82392899427642874, -291.2638794729775213, -343.5276183582624867 ) ) ;
#87807=CARTESIAN_POINT ( 'NONE',  ( -109.3021968867851825, -284.3703423667047332, -297.9083487441680518 ) ) ;
#87808=CARTESIAN_POINT ( 'NONE',  ( -111.2332909333861295, -270.9045546711798806, -253.6178120569185808 ) ) ;
#87809=CARTESIAN_POINT ( 'NONE',  ( -114.3549592388131089, -284.3543816369453907, -272.8471154920035815 ) ) ;
#87810=CARTESIAN_POINT ( 'NONE',  ( -110.9027961722705271, -280.3675749993185491, -283.1097993243005249 ) ) ;
#87811=CARTESIAN_POINT ( 'NONE',  ( -27.76965548478910861, -284.9713397811583491, -197.5908873549930433 ) ) ;
#87812=CARTESIAN_POINT ( 'NONE',  ( 37.10208548340217760, -285.6744022902821598, -279.8948927138080194 ) ) ;
#87813=CARTESIAN_POINT ( 'NONE',  ( -68.14823486232465655, -277.7915250317406617, -201.1280163957479488 ) ) ;
#87814=CARTESIAN_POINT ( 'NONE',  ( 202.9737475146022803, 296.4636489462809550, -68.70538243550777224 ) ) ;
#87815=CARTESIAN_POINT ( 'NONE',  ( -108.1544170132208791, -283.8225921268827392, -288.3485460695171128 ) ) ;
#87816=CARTESIAN_POINT ( 'NONE',  ( 38.27835170231957562, -282.9120234988077982, -282.6749376175422981 ) ) ;
#87817=CARTESIAN_POINT ( 'NONE',  ( -26.19061364126050151, -287.9722492800315194, -346.3115852793948193 ) ) ;
#87819=CARTESIAN_POINT ( 'NONE',  ( -37.10873657626705580, -278.6493676701351205, -346.5736879694478034 ) ) ;
#87820=CARTESIAN_POINT ( 'NONE',  ( -8.057802707929381469, -277.9916883904425049, -341.0559438451780352 ) ) ;
#87821=CARTESIAN_POINT ( 'NONE',  ( -7.997497824453166260, -280.2808996707357210, -203.5049603901559294 ) ) ;
#87822=CARTESIAN_POINT ( 'NONE',  ( -13.56486134083658435, -276.3422641958318309, -199.6044311005867939 ) ) ;
#87823=CARTESIAN_POINT ( 'NONE',  ( 32.23002095770841180, -293.9764070862005383, -303.4820113631884055 ) ) ;
#87824=CARTESIAN_POINT ( 'NONE',  ( 34.05526970268553555, -285.8438185008992605, -292.9499299655890923 ) ) ;
#87825=CARTESIAN_POINT ( 'NONE',  ( -50.44898863516970522, -293.4875930038789420, -195.2968828128720702 ) ) ;
#87826=CARTESIAN_POINT ( 'NONE',  ( 27.42474573565889173, -292.9396627380633049, -304.8138938082633445 ) ) ;
#87827=CARTESIAN_POINT ( 'NONE',  ( -36.99971132733521273, -294.7144391003879491, -343.3938889260370502 ) ) ;
#87828=CARTESIAN_POINT ( 'NONE',  ( -113.9418871746607351, -291.5850002449833482, -274.0899051016820067 ) ) ;
#87829=CARTESIAN_POINT ( 'NONE',  ( 35.66814197358649352, -282.2518914777602959, -274.0293088406166930 ) ) ;
#87830=CARTESIAN_POINT ( 'NONE',  ( -91.99311309434833106, -272.3536719687461414, -216.4533887270412151 ) ) ;
#87831=CARTESIAN_POINT ( 'NONE',  ( 20.50170990633611368, -288.8901530173038168, -321.0509953840277717 ) ) ;
#87832=CARTESIAN_POINT ( 'NONE',  ( 14.88466924481015674, -280.4648643266436920, -325.2492935840791688 ) ) ;
#87833=CARTESIAN_POINT ( 'NONE',  ( -12.22661540687209225, -289.0675544385782700, -343.1835667766744677 ) ) ;
#87834=CARTESIAN_POINT ( 'NONE',  ( -9.489252198181928222, -286.7596999542889193, -202.8470241216411694 ) ) ;
#87835=CARTESIAN_POINT ( 'NONE',  ( 184.9426652459831644, 263.7189940585919317, -153.2499980065188083 ) ) ;
#87836=CARTESIAN_POINT ( 'NONE',  ( 172.1150633234479130, 242.8691282751317715, -178.3881156067890856 ) ) ;
#87837=CARTESIAN_POINT ( 'NONE',  ( -111.3619333908369669, -270.6190337206908225, -283.6441699463446184 ) ) ;
#87839=CARTESIAN_POINT ( 'NONE',  ( -103.2809712672784315, -277.3200524974452605, -302.1740254065236400 ) ) ;
#87840=CARTESIAN_POINT ( 'NONE',  ( -108.5868433879396378, -277.6994155706966012, -253.0881438177620737 ) ) ;
#87841=CARTESIAN_POINT ( 'NONE',  ( -93.15391103601244538, -272.9438044071365539, -217.3254572891859482 ) ) ;
#87842=CARTESIAN_POINT ( 'NONE',  ( -110.3499187692159751, -272.5619384843310513, -283.8193449378834998 ) ) ;
#87843=CARTESIAN_POINT ( 'NONE',  ( -86.41232297056691891, -277.9613019756524750, -211.7201583158244773 ) ) ;
#87844=CARTESIAN_POINT ( 'NONE',  ( 16.85473502620386910, -296.0538781816921983, -323.6968519325373563 ) ) ;
#87846=CARTESIAN_POINT ( 'NONE',  ( -14.83339368574036321, -292.8441582102327061, -200.8530998648516004 ) ) ;
#87847=CARTESIAN_POINT ( 'NONE',  ( -109.8834447827226768, -273.8109361534544632, -245.2510503775759219 ) ) ;
#87848=CARTESIAN_POINT ( 'NONE',  ( -8.037149255852190421, -287.3450067515114483, -337.8134887777105746 ) ) ;
#87849=CARTESIAN_POINT ( 'NONE',  ( -94.07567327386276190, -273.9106882332212649, -218.4324347911523887 ) ) ;
#87850=CARTESIAN_POINT ( 'NONE',  ( -72.84873852150612095, -297.7343737101769534, -206.5782815056311961 ) ) ;
#87853=CARTESIAN_POINT ( 'NONE',  ( -61.60874427780643714, -281.6595886891419696, -198.7487871562420594 ) ) ;
#87854=CARTESIAN_POINT ( 'NONE',  ( -108.9115236253497727, -279.8410365807625340, -254.4295215951917157 ) ) ;
#87855=CARTESIAN_POINT ( 'NONE',  ( -106.6426046061193347, -279.9074602337205988, -301.6556943183560406 ) ) ;
#87856=CARTESIAN_POINT ( 'NONE',  ( -51.67756258524116220, -272.3454429611390424, -198.0233580618600229 ) ) ;
#87859=CARTESIAN_POINT ( 'NONE',  ( -66.07165578414669938, -279.8320861067056740, -203.2386890866297620 ) ) ;
#87860=CARTESIAN_POINT ( 'NONE',  ( 27.51802948873118737, -276.8971844221867400, -311.6592441789029522 ) ) ;
#87861=CARTESIAN_POINT ( 'NONE',  ( 0.07202887891175330237, -278.5547186161049353, -335.4216775580864578 ) ) ;
#87862=CARTESIAN_POINT ( 'NONE',  ( -41.37165895666818471, -275.6766613382840774, -346.6786536304115316 ) ) ;
#87865=CARTESIAN_POINT ( 'NONE',  ( 25.36740913513376228, -284.0940114570599349, -312.1459767013844839 ) ) ;
#87866=CARTESIAN_POINT ( 'NONE',  ( -52.39302613426399802, -291.0517364691212379, -198.7126004384512612 ) ) ;
#87867=CARTESIAN_POINT ( 'NONE',  ( -30.88413497854260825, -285.4803013588013414, -193.7213920461151702 ) ) ;
#87869=CARTESIAN_POINT ( 'NONE',  ( -102.6761366201529881, -282.3233178885338930, -305.2464769691491142 ) ) ;
#87870=CARTESIAN_POINT ( 'NONE',  ( -21.27712114649834874, -281.4169056330804892, -342.2279213674067933 ) ) ;
#87871=CARTESIAN_POINT ( 'NONE',  ( 33.83691006298187887, -282.5215504107740685, -252.4009963932691960 ) ) ;
#87873=CARTESIAN_POINT ( 'NONE',  ( -0.7774042487873865648, -280.9747885032955423, -337.2301645685524818 ) ) ;
#87874=CARTESIAN_POINT ( 'NONE',  ( -2.863612568200582853, -296.5965519383203741, -336.9663890208366865 ) ) ;
#87875=CARTESIAN_POINT ( 'NONE',  ( -92.58994931416631857, -287.2637938616313136, -219.3175681747101464 ) ) ;
#87877=CARTESIAN_POINT ( 'NONE',  ( -89.80406003569667917, -293.2393824680316925, -215.9100361501383816 ) ) ;
#87878=CARTESIAN_POINT ( 'NONE',  ( -10.56310195994404744, -274.7026527240260521, -340.4175761360866090 ) ) ;
#87879=CARTESIAN_POINT ( 'NONE',  ( 3.086462501390835111, -287.7214100702919382, -335.7666434807213136 ) ) ;
#87880=CARTESIAN_POINT ( 'NONE',  ( 35.00472939265675620, -291.7618352757755247, -255.7859832433047131 ) ) ;
#87881=CARTESIAN_POINT ( 'NONE',  ( -78.92473631777671983, -276.3102529597454122, -331.0209059810728149 ) ) ;
#87882=CARTESIAN_POINT ( 'NONE',  ( -111.4764145802917739, -294.6416401280158084, -274.2224119298620622 ) ) ;
#87883=CARTESIAN_POINT ( 'NONE',  ( -78.43638957310510307, -290.9329033703104983, -331.3524169317448695 ) ) ;
#87886=CARTESIAN_POINT ( 'NONE',  ( -95.99106007723788991, -294.3693075224383620, -319.1970165281655341 ) ) ;
#87887=CARTESIAN_POINT ( 'NONE',  ( 33.08310672844088884, -289.4435265653527836, -292.5946040085141817 ) ) ;
#87888=CARTESIAN_POINT ( 'NONE',  ( -105.0903484159690464, -289.2422833965050017, -235.8344908930976089 ) ) ;
#87890=CARTESIAN_POINT ( 'NONE',  ( -73.82141028047767861, -290.9719447049801602, -334.2865637977051847 ) ) ;
#87892=CARTESIAN_POINT ( 'NONE',  ( -58.72658632304552384, -290.1386151735616750, -340.3803734966105594 ) ) ;
#87894=CARTESIAN_POINT ( 'NONE',  ( 28.56994127070791833, -289.2683969637597556, -309.3952600369004244 ) ) ;
#87895=CARTESIAN_POINT ( 'NONE',  ( -50.62440045209152828, -277.9034137490165222, -196.1858075877599674 ) ) ;
#87896=CARTESIAN_POINT ( 'NONE',  ( -17.00166326942441941, -280.6411188445425182, -196.1180900807452190 ) ) ;
#87898=CARTESIAN_POINT ( 'NONE',  ( -84.55061755013238667, -279.0890620244917955, -209.4901913336462655 ) ) ;
#87899=CARTESIAN_POINT ( 'NONE',  ( -22.02722297091859005, -284.2480557307476943, -196.8880092554559553 ) ) ;
#87901=CARTESIAN_POINT ( 'NONE',  ( -7.481216490278900899, -278.5874375800243001, -202.3823900990478535 ) ) ;
#87902=CARTESIAN_POINT ( 'NONE',  ( -0.1462403245302671961, -280.5572363392818716, -335.5027392383176448 ) ) ;
#87903=CARTESIAN_POINT ( 'NONE',  ( 65.57626948303558834, 46.04035151990646568, -315.5245225855154558 ) ) ;
#87904=CARTESIAN_POINT ( 'NONE',  ( -102.8067277124654737, -277.5490806789696876, -231.0533460065475992 ) ) ;
#87906=CARTESIAN_POINT ( 'NONE',  ( -93.28324136726352833, -298.7488908410369390, -222.3703382689367345 ) ) ;
#87907=CARTESIAN_POINT ( 'NONE',  ( -93.21579149257897257, -282.7524505627250733, -322.9120638260972100 ) ) ;
#87908=CARTESIAN_POINT ( 'NONE',  ( -93.04335610944514201, -274.0283414755382978, -222.9083780918271316 ) ) ;
#87909=CARTESIAN_POINT ( 'NONE',  ( -100.7299780848046851, -274.5449262412594749, -227.5991901259323811 ) ) ;
#87910=CARTESIAN_POINT ( 'NONE',  ( 9.674423792316273918, -276.0506426022662367, -326.2321442679535153 ) ) ;
#87911=CARTESIAN_POINT ( 'NONE',  ( -50.80591882042548235, -297.2243425790355218, -344.1426567367664120 ) ) ;
#87912=CARTESIAN_POINT ( 'NONE',  ( -99.02786209136434081, -290.1054647251472716, -316.4678148511616769 ) ) ;
#87913=CARTESIAN_POINT ( 'NONE',  ( -35.34902974488176142, -278.1567995710110495, -194.8145030839573622 ) ) ;
#87914=CARTESIAN_POINT ( 'NONE',  ( -103.2147430340040017, -290.9070216713524815, -230.3867501558528659 ) ) ;
#87915=CARTESIAN_POINT ( 'NONE',  ( -63.91742271541528453, -288.4660337244906714, -338.6587187799153753 ) ) ;
#87916=CARTESIAN_POINT ( 'NONE',  ( 31.49900719815166994, -291.1625969176334365, -240.5960770669717022 ) ) ;
#87919=CARTESIAN_POINT ( 'NONE',  ( -91.71476639531482533, -290.7578320876427256, -221.5411972717067215 ) ) ;
#87921=CARTESIAN_POINT ( 'NONE',  ( 14.08034650069721394, -287.6942441104267800, -213.2933802456728927 ) ) ;
#87922=CARTESIAN_POINT ( 'NONE',  ( 7.450504543161046378, -290.9090924074130839, -326.4764044574609443 ) ) ;
#87923=CARTESIAN_POINT ( 'NONE',  ( -76.97106242482884397, -294.6277348318757277, -336.1674232490917120 ) ) ;
#87924=CARTESIAN_POINT ( 'NONE',  ( 33.11834065751056499, -283.2506969315764422, -300.3072340868965853 ) ) ;
#87925=CARTESIAN_POINT ( 'NONE',  ( -103.4845654490978006, -284.8040106972706553, -239.3524400010108195 ) ) ;
#87926=CARTESIAN_POINT ( 'NONE',  ( 31.57499046054697445, -276.5291850193854657, -244.8320514969676083 ) ) ;
#87927=CARTESIAN_POINT ( 'NONE',  ( -15.12683528741805006, -292.7832932191679447, -341.6779998885816667 ) ) ;
#87928=CARTESIAN_POINT ( 'NONE',  ( -34.00736838304376164, -272.8899445245073139, -197.0398200030965086 ) ) ;
#87931=CARTESIAN_POINT ( 'NONE',  ( -41.94853952484770332, -294.7752964004404816, -347.2543800968483083 ) ) ;
#87932=CARTESIAN_POINT ( 'NONE',  ( -49.68389497884351869, -287.8138363986287800, -196.8988984098576225 ) ) ;
#87933=CARTESIAN_POINT ( 'NONE',  ( -106.2416603535695003, -298.0660356230430352, -236.6819257446770735 ) ) ;
#87934=CARTESIAN_POINT ( 'NONE',  ( -4.556271929034998003, -287.1474464090086940, -205.0234690629803822 ) ) ;
#87935=CARTESIAN_POINT ( 'NONE',  ( -104.7746302762587334, -277.1347619277786407, -307.0438134120429936 ) ) ;
#87936=CARTESIAN_POINT ( 'NONE',  ( -47.60974176277625247, -295.8308449965302316, -346.5705669201018964 ) ) ;
#87937=CARTESIAN_POINT ( 'NONE',  ( -86.59965555868208753, -287.8673341026253638, -327.9970452266349525 ) ) ;
#87938=CARTESIAN_POINT ( 'NONE',  ( -0.7124965584789343387, -294.9125224610830855, -338.0815808444419304 ) ) ;
#87939=CARTESIAN_POINT ( 'NONE',  ( -20.07127747165285214, -292.6134109575561979, -199.3594156553337200 ) ) ;
#87942=CARTESIAN_POINT ( 'NONE',  ( 202.8071895515903122, 291.9636489450776367, -53.99999999998529887 ) ) ;
#87943=CARTESIAN_POINT ( 'NONE',  ( 22.43654311266901757, -288.4316029728053081, -222.9138358805863049 ) ) ;
#87944=CARTESIAN_POINT ( 'NONE',  ( -55.63300648810263738, -280.7666405000205145, -350.3538533559490702 ) ) ;
#87946=CARTESIAN_POINT ( 'NONE',  ( -106.4697971116899708, -283.1472905864703762, -294.9158951522919097 ) ) ;
#87947=CARTESIAN_POINT ( 'NONE',  ( -68.62345302996259022, -279.0003322675260051, -200.0988715810434257 ) ) ;
#87948=CARTESIAN_POINT ( 'NONE',  ( 8.239338077805580696, -282.6770541049942835, -210.9457823598843902 ) ) ;
#87949=CARTESIAN_POINT ( 'NONE',  ( 195.6275670422409121, 276.7432394079091864, -125.1359736961868094 ) ) ;
#87950=CARTESIAN_POINT ( 'NONE',  ( -85.13016272798500950, -283.9816499904911211, -210.7383946833309096 ) ) ;
#87951=CARTESIAN_POINT ( 'NONE',  ( -40.03424356761348690, -287.1659660441360984, -344.8029690430848291 ) ) ;
#87952=CARTESIAN_POINT ( 'NONE',  ( -70.87772589190122119, -275.4748417354322214, -202.4226129911748444 ) ) ;
#87953=CARTESIAN_POINT ( 'NONE',  ( -35.82025859689427705, -298.5640525009145563, -197.2994475690733225 ) ) ;
#87954=CARTESIAN_POINT ( 'NONE',  ( -69.95788853338572721, -294.1759199753086023, -336.2202687019762379 ) ) ;
#87955=CARTESIAN_POINT ( 'NONE',  ( -110.4553604842015062, -279.5056089338852416, -246.3654859261420711 ) ) ;
#87956=CARTESIAN_POINT ( 'NONE',  ( -6.276626249304853467, -276.6322962131042118, -336.4351709322590978 ) ) ;
#87957=CARTESIAN_POINT ( 'NONE',  ( -70.01263078546087115, -274.7115398422857311, -200.9630256873461178 ) ) ;
#87958=CARTESIAN_POINT ( 'NONE',  ( -70.18118318084478346, -276.3950422615041589, -339.6796170912918456 ) ) ;
#87959=CARTESIAN_POINT ( 'NONE',  ( 201.7240241516113883, 293.7293971981039249, -83.18315247050524874 ) ) ;
#87960=CARTESIAN_POINT ( 'NONE',  ( 35.71074788677532297, -273.3332557589060912, -253.3251306200568536 ) ) ;
#87962=CARTESIAN_POINT ( 'NONE',  ( -113.0207262607261498, -298.1115689942610629, -259.7168405879997977 ) ) ;
#87963=CARTESIAN_POINT ( 'NONE',  ( -4.829096099716510437, -276.9805209788416391, -202.7746430608542312 ) ) ;
#87967=CARTESIAN_POINT ( 'NONE',  ( 0.3156950102680667891, -287.6458032309157602, -207.4040360855865401 ) ) ;
#87968=CARTESIAN_POINT ( 'NONE',  ( -111.5308084045867645, -286.1040646807946359, -286.7912802056800388 ) ) ;
#87969=CARTESIAN_POINT ( 'NONE',  ( -71.21810162729639160, -284.9410305949313624, -205.5824016482220031 ) ) ;
#87970=CARTESIAN_POINT ( 'NONE',  ( -100.1378508476021949, -277.4820002764039941, -231.4940445704830267 ) ) ;
#87971=CARTESIAN_POINT ( 'NONE',  ( -96.89878241031334483, -285.8012777371054653, -314.6761203247119738 ) ) ;
#87972=CARTESIAN_POINT ( 'NONE',  ( -51.94600347293249598, -278.3418665363128071, -198.0771736227187887 ) ) ;
#87973=CARTESIAN_POINT ( 'NONE',  ( 22.72699112690552425, -277.2164240022154900, -312.4718365316028326 ) ) ;
#87974=CARTESIAN_POINT ( 'NONE',  ( -24.59185279622966291, -274.7114757930288533, -198.3690263999752119 ) ) ;
#87976=CARTESIAN_POINT ( 'NONE',  ( 33.42122297475751935, -282.7384379602993931, -300.4431182021271525 ) ) ;
#87977=CARTESIAN_POINT ( 'NONE',  ( -37.30797974140362072, -283.5440486210492850, -347.3126272967377872 ) ) ;
#87981=CARTESIAN_POINT ( 'NONE',  ( -2.807406897773097487, -288.3640664758796106, -202.9100554294749372 ) ) ;
#87982=CARTESIAN_POINT ( 'NONE',  ( -107.2873572870556416, -288.8373857931518387, -301.4899233774992808 ) ) ;
#87983=CARTESIAN_POINT ( 'NONE',  ( -108.9350283906195642, -295.9484065043043302, -255.2345005460501852 ) ) ;
#87984=CARTESIAN_POINT ( 'NONE',  ( -19.40249083884732428, -291.6255195040851618, -195.5300499481670613 ) ) ;
#87986=CARTESIAN_POINT ( 'NONE',  ( 12.61169566093211181, -286.8207983584915723, -324.6094593921056344 ) ) ;
#87987=CARTESIAN_POINT ( 'NONE',  ( -61.46516422921862954, -287.9464802710733693, -339.8840163422664773 ) ) ;
#87988=CARTESIAN_POINT ( 'NONE',  ( -65.25838830001563906, -286.8841930095118187, -202.4263146863197562 ) ) ;
#87989=CARTESIAN_POINT ( 'NONE',  ( -111.1034233778913887, -276.3768176456035235, -284.0041622790973292 ) ) ;
#87990=CARTESIAN_POINT ( 'NONE',  ( 36.36535705571708377, -286.1965563239162407, -289.6927019466888851 ) ) ;
#87991=CARTESIAN_POINT ( 'NONE',  ( 37.36010764197031619, -289.4593949982132131, -263.1242357017363815 ) ) ;
#87992=CARTESIAN_POINT ( 'NONE',  ( 4.514799762249682047, -286.4885950582082046, -332.7955783505865384 ) ) ;
#87993=CARTESIAN_POINT ( 'NONE',  ( -104.3236853509115463, -285.0961815561117874, -299.9723000431780520 ) ) ;
#87994=CARTESIAN_POINT ( 'NONE',  ( -70.12177187658431876, -293.6214269528587124, -202.7187102213882497 ) ) ;
#87997=CARTESIAN_POINT ( 'NONE',  ( -97.95226509816951932, -299.0840389123143268, -225.2210749450559888 ) ) ;
#87998=CARTESIAN_POINT ( 'NONE',  ( -39.69620903541504475, -279.2190284270445204, -197.2249899774763833 ) ) ;
#87999=CARTESIAN_POINT ( 'NONE',  ( 35.58915388519211120, -279.7773365921232198, -287.9111417896199896 ) ) ;
#88000=CARTESIAN_POINT ( 'NONE',  ( 38.16845473548401202, -292.5710351991092466, -256.1352495251503569 ) ) ;
#88001=CARTESIAN_POINT ( 'NONE',  ( -74.76669074656729208, -271.7869274108691684, -206.4476740750432668 ) ) ;
#88002=CARTESIAN_POINT ( 'NONE',  ( -32.34790973844188500, -275.0686768468325454, -344.6843819489247949 ) ) ;
#88003=CARTESIAN_POINT ( 'NONE',  ( -86.80963664459045503, -297.0729216642727692, -324.7133647965742966 ) ) ;
#88005=CARTESIAN_POINT ( 'NONE',  ( -46.79001135833403424, -272.5091478152562559, -194.5367438878168116 ) ) ;
#88006=CARTESIAN_POINT ( 'NONE',  ( -110.9920956273559653, -294.5543349724370614, -289.1111225983144095 ) ) ;
#88008=CARTESIAN_POINT ( 'NONE',  ( 32.91470747113712036, -295.2652479807409236, -292.2565994486166119 ) ) ;
#88010=CARTESIAN_POINT ( 'NONE',  ( -84.57457205418812407, -296.5248457773866448, -326.2994218480039308 ) ) ;
#88012=CARTESIAN_POINT ( 'NONE',  ( -57.29559367141229842, -283.8161574905348630, -197.6416323532493493 ) ) ;
#88013=CARTESIAN_POINT ( 'NONE',  ( -110.3841182491784991, -296.5376149731446276, -271.4631167961459823 ) ) ;
#88014=CARTESIAN_POINT ( 'NONE',  ( -76.75789514397068558, -283.5641499417304772, -336.5694682708411847 ) ) ;
#88015=CARTESIAN_POINT ( 'NONE',  ( 32.24941778125134562, -283.8555796135488549, -299.9293527373164352 ) ) ;
#88016=CARTESIAN_POINT ( 'NONE',  ( -64.53574935218415476, -285.3734318282904496, -198.3314841712942211 ) ) ;
#88017=CARTESIAN_POINT ( 'NONE',  ( -0.3282714067713123907, -290.5452906432827263, -205.3075611051781948 ) ) ;
#88018=CARTESIAN_POINT ( 'NONE',  ( -95.95921662488163406, -276.6952119285918457, -223.5744983911110353 ) ) ;
#88020=CARTESIAN_POINT ( 'NONE',  ( 7.179900938095929774, -285.4687564448618673, -211.9448784554365659 ) ) ;
#88021=CARTESIAN_POINT ( 'NONE',  ( -69.24132009131211873, -288.3823767429618670, -340.1171996956661587 ) ) ;
#88023=CARTESIAN_POINT ( 'NONE',  ( -113.6236803329639429, -280.0333115146350451, -265.9265055395104014 ) ) ;
#88024=CARTESIAN_POINT ( 'NONE',  ( -34.93302407509652596, -293.0421440463298381, -345.6778165645779382 ) ) ;
#88025=CARTESIAN_POINT ( 'NONE',  ( 33.78194858457152350, -281.0007626259030644, -253.8228568684648963 ) ) ;
#88026=CARTESIAN_POINT ( 'NONE',  ( 19.53111540539381608, -294.4252453836471091, -322.3471917137055698 ) ) ;
#88028=CARTESIAN_POINT ( 'NONE',  ( -83.36039144849959825, -281.4221282135485467, -211.0730805485362396 ) ) ;
#88029=CARTESIAN_POINT ( 'NONE',  ( -38.35754238776203806, -294.1239411967820843, -343.5893674043023793 ) ) ;
#88031=CARTESIAN_POINT ( 'NONE',  ( -36.88564129984808204, -296.0577044583180850, -195.3612647501385595 ) ) ;
#88035=CARTESIAN_POINT ( 'NONE',  ( 14.45878185895233692, -282.7644997205793516, -216.5438152142829438 ) ) ;
#88036=CARTESIAN_POINT ( 'NONE',  ( -93.13344359532653982, -295.3897704676152216, -317.5532668033202413 ) ) ;
#88038=CARTESIAN_POINT ( 'NONE',  ( -69.91165696735023971, -280.9809262143061233, -337.9199732462171255 ) ) ;
#88039=CARTESIAN_POINT ( 'NONE',  ( -13.10371249219858925, -273.5564123017754810, -197.4455587681865723 ) ) ;
#88041=CARTESIAN_POINT ( 'NONE',  ( -94.10562526046624043, -289.7362468628363672, -316.2616278719199272 ) ) ;
#88043=CARTESIAN_POINT ( 'NONE',  ( -67.60858399614113523, -281.1678115959601882, -203.1564324437556763 ) ) ;
#88044=CARTESIAN_POINT ( 'NONE',  ( -74.69570621828421508, -275.1466549277791955, -206.6535127026903353 ) ) ;
#88045=CARTESIAN_POINT ( 'NONE',  ( -3.232469343243530080, -284.2094172916588946, -338.5151890446434209 ) ) ;
#88046=CARTESIAN_POINT ( 'NONE',  ( -72.30542045162339093, -278.3734765558481286, -205.8268730681629108 ) ) ;
#88047=CARTESIAN_POINT ( 'NONE',  ( 8.831183281731817658, -278.4196222314847660, -329.5294736393781818 ) ) ;
#88049=CARTESIAN_POINT ( 'NONE',  ( -34.10107067241351331, -273.9251751815434659, -193.4293408988897340 ) ) ;
#88050=CARTESIAN_POINT ( 'NONE',  ( -5.446378197264083454, -294.3951994222476856, -203.0863604086629834 ) ) ;
#88051=DIRECTION ( 'NONE',  ( 0.000000000000000000, 0.000000000000000000, 1.000000000000000000 ) ) ;
#88053=CARTESIAN_POINT ( 'NONE',  ( -41.89539172292137437, -293.2484082096262910, -346.0405049937615445 ) ) ;
#88054=CARTESIAN_POINT ( 'NONE',  ( -97.89067727954578402, -272.6287297398000078, -229.3831018076481598 ) ) ;
#88056=CARTESIAN_POINT ( 'NONE',  ( 16.98228717613609362, -294.3288933417796329, -216.6993093001383386 ) ) ;
#88057=CARTESIAN_POINT ( 'NONE',  ( -4.829096099716510437, -282.9805209788416391, -202.7746430608542312 ) ) ;
#88058=CARTESIAN_POINT ( 'NONE',  ( -3.794977272724276318, -288.4959754479165213, -203.4683245288587443 ) ) ;
#88059=CARTESIAN_POINT ( 'NONE',  ( -13.21789937088826150, -274.7380510615967637, -341.2539243625914764 ) ) ;
#88060=CARTESIAN_POINT ( 'NONE',  ( 29.33093044711479180, -277.9138853626754440, -303.5844146361203002 ) ) ;
#88061=CARTESIAN_POINT ( 'NONE',  ( 36.73076434529306766, -291.5299507287904817, -262.4731581731098231 ) ) ;
#88062=CARTESIAN_POINT ( 'NONE',  ( -110.5438516166715459, -280.6617613517578889, -250.7725339633181534 ) ) ;
#88064=CARTESIAN_POINT ( 'NONE',  ( -40.23944534481395152, -282.7562954043267496, -343.3247428890520041 ) ) ;
#88065=CARTESIAN_POINT ( 'NONE',  ( -64.64518714521443599, -280.7836883358521618, -198.6391335974570609 ) ) ;
#88067=CARTESIAN_POINT ( 'NONE',  ( -47.22043294360042864, -281.9699420839394293, -346.3243943458421654 ) ) ;
#88068=CARTESIAN_POINT ( 'NONE',  ( 20.65039207745597594, -277.1753149104871454, -320.6775120918483140 ) ) ;
#88070=CARTESIAN_POINT ( 'NONE',  ( 23.07194617520410063, -276.4442403298035060, -223.7254904445416344 ) ) ;
#88071=CARTESIAN_POINT ( 'NONE',  ( -105.5795714935544112, -292.8376638359844719, -285.9686137636504668 ) ) ;
#88074=CARTESIAN_POINT ( 'NONE',  ( -100.1356641409920059, -299.1065787196612291, -229.2558880299098689 ) ) ;
#88075=CARTESIAN_POINT ( 'NONE',  ( -72.78841978645263566, -292.6509560028214878, -206.1343243186854863 ) ) ;
#88076=CARTESIAN_POINT ( 'NONE',  ( -73.66393723770808322, -275.5568203661385382, -335.5873427672989351 ) ) ;
#88077=CARTESIAN_POINT ( 'NONE',  ( -8.595433050809544895, -290.4412316765368587, -340.7145625764255215 ) ) ;
#88078=CARTESIAN_POINT ( 'NONE',  ( -85.99068765710171647, -290.7055391803672819, -215.7295545633712663 ) ) ;
#88079=CARTESIAN_POINT ( 'NONE',  ( 39.64079791239883832, -287.0747689296518388, -271.5565952383105355 ) ) ;
#88081=CARTESIAN_POINT ( 'NONE',  ( -53.88864543901411253, -281.6678207017998261, -342.3348377082150478 ) ) ;
#88082=CARTESIAN_POINT ( 'NONE',  ( -72.93055549288244777, -291.3894515667271321, -335.5094015790838284 ) ) ;
#88083=CARTESIAN_POINT ( 'NONE',  ( -102.3922678062164522, -282.5632985167258653, -305.0982545796017575 ) ) ;
#88084=CARTESIAN_POINT ( 'NONE',  ( -39.73395180052004605, -281.3366925667725695, -196.8943062102937631 ) ) ;
#88085=CARTESIAN_POINT ( 'NONE',  ( -106.2968676754041439, -291.0575067044758839, -304.2162379658692544 ) ) ;
#88086=CARTESIAN_POINT ( 'NONE',  ( -110.4534897544638881, -279.0407669068110863, -270.6445443924029064 ) ) ;
#88087=CARTESIAN_POINT ( 'NONE',  ( -19.46446794593252960, -291.0719460744298317, -195.8189035277109724 ) ) ;
#88088=CARTESIAN_POINT ( 'NONE',  ( 34.69927799345143171, -288.0163770757100679, -243.6355442475868074 ) ) ;
#88089=CARTESIAN_POINT ( 'NONE',  ( 38.61525139615243063, -288.2018822288491151, -282.9354233038869211 ) ) ;
#88090=CARTESIAN_POINT ( 'NONE',  ( -39.97604399891438476, -286.1848131685628118, -197.4086660916569258 ) ) ;
#88091=EDGE_LOOP ( 'NONE', ( #48960, #80585 ) ) ;
#88093=CARTESIAN_POINT ( 'NONE',  ( 28.39203342393819440, -294.9150701284098659, -232.6864348158137261 ) ) ;
#88094=CARTESIAN_POINT ( 'NONE',  ( -99.61691144699085498, -294.6435072871005900, -314.8924308792064721 ) ) ;
#88095=CARTESIAN_POINT ( 'NONE',  ( 19.35616632030332696, -275.2653556777614767, -316.7355984258047670 ) ) ;
#88096=CARTESIAN_POINT ( 'NONE',  ( -98.14825962218955624, -296.5302480525601254, -223.2667873263114302 ) ) ;
#88097=CARTESIAN_POINT ( 'NONE',  ( 33.78080959018988239, -292.2850808385719574, -289.7040323429512227 ) ) ;
#88098=CARTESIAN_POINT ( 'NONE',  ( -109.5858086981793633, -294.5827131127281291, -286.4472235874768558 ) ) ;
#88099=AXIS2_PLACEMENT_3D ( 'NONE', #5813, #19083, #91494 ) ;
#88100=CARTESIAN_POINT ( 'NONE',  ( -52.46650105825904120, -293.0593217127251364, -198.4871328024764523 ) ) ;
#88101=CARTESIAN_POINT ( 'NONE',  ( 10.50361382554200063, -295.4525027874370267, -325.9043624448160585 ) ) ;
#88104=CARTESIAN_POINT ( 'NONE',  ( 32.73293801919767532, -291.9049436001784557, -297.5562188825014687 ) ) ;
#88105=CARTESIAN_POINT ( 'NONE',  ( -96.75263409797366876, -297.9249393878914702, -316.1566897943395702 ) ) ;
#88106=CARTESIAN_POINT ( 'NONE',  ( -110.3562042000021108, -291.4105568231588563, -276.6620431624808703 ) ) ;
#88108=CARTESIAN_POINT ( 'NONE',  ( -42.38694992656297700, -295.4508147315298174, -343.2077578588712186 ) ) ;
#88110=CARTESIAN_POINT ( 'NONE',  ( -79.28920299328233057, -279.5947256136594206, -333.0243484806517245 ) ) ;
#88111=CARTESIAN_POINT ( 'NONE',  ( -111.9172554601288567, -277.4519923052437775, -253.2794078170714158 ) ) ;
#88113=CARTESIAN_POINT ( 'NONE',  ( -66.18128497136308397, -273.0330382519287582, -199.0616873903806265 ) ) ;
#88114=CARTESIAN_POINT ( 'NONE',  ( 22.96444719138651891, -280.2309726238613052, -314.0233138409413982 ) ) ;
#88115=CARTESIAN_POINT ( 'NONE',  ( -112.5133435743650097, -276.7943531801821564, -282.8376735028777489 ) ) ;
#88116=CARTESIAN_POINT ( 'NONE',  ( -108.7986888273022004, -276.8544628302996671, -246.8738483912092363 ) ) ;
#88117=CARTESIAN_POINT ( 'NONE',  ( -63.23765619511080871, -296.3925755081279476, -201.5276133702380434 ) ) ;
#88120=CARTESIAN_POINT ( 'NONE',  ( -111.3055743514985636, -288.7573173876669443, -255.8804036379154638 ) ) ;
#88121=CARTESIAN_POINT ( 'NONE',  ( -114.2513007961944140, -290.5055026580545814, -274.0911749622030129 ) ) ;
#88122=CARTESIAN_POINT ( 'NONE',  ( -4.647123075323000840, -276.4819619285366343, -202.6631852457198875 ) ) ;
#88123=CARTESIAN_POINT ( 'NONE',  ( -76.13990737606391690, -295.5326814295020199, -206.3109919767010751 ) ) ;
#88124=CARTESIAN_POINT ( 'NONE',  ( -63.86588771210455207, -282.5865781149620943, -342.4764859241964814 ) ) ;
#88126=CARTESIAN_POINT ( 'NONE',  ( 37.14009450132499524, -279.6704666828625818, -279.5883913115331438 ) ) ;
#88127=CIRCLE ( 'NONE', #41212, 2.336627660646517501 ) ;
#88129=CARTESIAN_POINT ( 'NONE',  ( 15.17026737379739387, -291.6085045964363758, -219.0084496902107674 ) ) ;
#88130=CARTESIAN_POINT ( 'NONE',  ( -109.5617619924906592, -282.9152455127450025, -253.1271530884613981 ) ) ;
#88133=CARTESIAN_POINT ( 'NONE',  ( 29.27433581912985971, -291.0959216691383631, -235.9038342759135674 ) ) ;
#88134=CARTESIAN_POINT ( 'NONE',  ( -96.72473094528029947, -279.5445122500848925, -314.2011936995983206 ) ) ;
#88135=CARTESIAN_POINT ( 'NONE',  ( 8.980949324553606061, -283.6372816363866605, -331.3711242534291728 ) ) ;
#88136=CARTESIAN_POINT ( 'NONE',  ( -8.222485250906748533, -272.5102064271576410, -200.5819330462015841 ) ) ;
#88137=CARTESIAN_POINT ( 'NONE',  ( -85.72614845339728618, -285.3604186175128916, -215.6314559081591256 ) ) ;
#88138=CARTESIAN_POINT ( 'NONE',  ( 34.69443761783420399, -276.7798228385889843, -255.2607302509971134 ) ) ;
#88139=CARTESIAN_POINT ( 'NONE',  ( -69.31276912897160969, -278.2866883597445167, -336.1811584178219618 ) ) ;
#88140=ADVANCED_FACE ( 'NONE', ( #11798 ), #53957, .T. ) ;
#88141=CARTESIAN_POINT ( 'NONE',  ( -90.98498959451472956, -285.8140612892287322, -322.7767467906639354 ) ) ;
#88145=CARTESIAN_POINT ( 'NONE',  ( -113.6529222429083887, -296.2520716419392102, -281.0277591448146381 ) ) ;
#88146=CARTESIAN_POINT ( 'NONE',  ( 7.904344611423861799, -288.6532118800534477, -210.9271306806662380 ) ) ;
#88148=CARTESIAN_POINT ( 'NONE',  ( 40.65961533371913106, -284.8380690714489560, -252.5904736702033802 ) ) ;
#88149=CARTESIAN_POINT ( 'NONE',  ( -69.81891132980183556, -278.5548227276381681, -200.8721641875049215 ) ) ;
#88150=CARTESIAN_POINT ( 'NONE',  ( -55.97325112671786229, -290.2161168959786437, -196.4196302003576307 ) ) ;
#88151=CARTESIAN_POINT ( 'NONE',  ( -109.6126816646767423, -286.2605644282862727, -255.9523365685023464 ) ) ;
#88152=CARTESIAN_POINT ( 'NONE',  ( -77.38873885318605517, -281.2674942412294854, -208.0568696274944216 ) ) ;
#88153=CARTESIAN_POINT ( 'NONE',  ( 38.76601831549815813, -288.8845994184816277, -262.9958655472564146 ) ) ;
#88154=CARTESIAN_POINT ( 'NONE',  ( -10.22964350021393010, -284.6985922702266976, -340.3442601395365728 ) ) ;
#88155=CARTESIAN_POINT ( 'NONE',  ( -28.59892865729863942, -277.1109960324056374, -346.9167453941711869 ) ) ;
#88156=CARTESIAN_POINT ( 'NONE',  ( -108.9434146600346480, -270.8350489116736526, -248.4301281355177196 ) ) ;
#88157=CARTESIAN_POINT ( 'NONE',  ( -22.56410032880094718, -280.0694853920627452, -194.7382011148541494 ) ) ;
#88159=CARTESIAN_POINT ( 'NONE',  ( -47.49284973818976141, -299.8424327094240311, -196.5642795176598838 ) ) ;
#88161=CARTESIAN_POINT ( 'NONE',  ( 35.78497577281001440, -278.2662352645559167, -287.0191576251351080 ) ) ;
#88162=CARTESIAN_POINT ( 'NONE',  ( 13.30597666025241388, -272.9885491447457753, -213.6446295069706025 ) ) ;
#88165=CARTESIAN_POINT ( 'NONE',  ( -110.2195865913370199, -278.1280386710591870, -265.1840429234287058 ) ) ;
#88167=CARTESIAN_POINT ( 'NONE',  ( 36.85797481993009228, -276.9966972091705770, -289.3983698169153627 ) ) ;
#88168=CARTESIAN_POINT ( 'NONE',  ( 39.40591682538859430, -280.5697338323745385, -267.0794283067742185 ) ) ;
#88169=CARTESIAN_POINT ( 'NONE',  ( -71.62246852129017327, -291.2716265218506919, -335.9711885992347788 ) ) ;
#88170=CARTESIAN_POINT ( 'NONE',  ( -29.17167597755265973, -299.6727988630092341, -194.0523781336487446 ) ) ;
#88171=CARTESIAN_POINT ( 'NONE',  ( -80.41450008066351529, -298.6880337901230291, -206.9511208581930362 ) ) ;
#88172=CARTESIAN_POINT ( 'NONE',  ( -6.538296825703257653, -294.4577616521149821, -202.1615668486769550 ) ) ;
#88173=CARTESIAN_POINT ( 'NONE',  ( 6.649781761084901710, -280.4522460333596996, -330.8985274488123878 ) ) ;
#88175=CARTESIAN_POINT ( 'NONE',  ( 31.67866088699393501, -283.8384726241913540, -298.2448759950679573 ) ) ;
#88176=CARTESIAN_POINT ( 'NONE',  ( -75.08374230413420491, -271.5672118961417709, -205.9010585980348935 ) ) ;
#88177=CARTESIAN_POINT ( 'NONE',  ( -109.2293572722669097, -286.4744047880150788, -245.0904795891546541 ) ) ;
#88178=CARTESIAN_POINT ( 'NONE',  ( -73.71021151142527117, -288.4674053433036534, -334.0274374160937896 ) ) ;
#88179=CARTESIAN_POINT ( 'NONE',  ( 162.5749643528775152, 219.4908287816205927, -205.1158602168718232 ) ) ;
#88181=CARTESIAN_POINT ( 'NONE',  ( -65.24886689772108639, -287.9844206219984812, -341.5492815931301038 ) ) ;
#88182=CARTESIAN_POINT ( 'NONE',  ( 33.72068467352190169, -287.4404327710979032, -287.1606701546808722 ) ) ;
#88184=CARTESIAN_POINT ( 'NONE',  ( -113.1838493221684701, -285.7790947585094727, -258.6324309697760100 ) ) ;
#88186=CARTESIAN_POINT ( 'NONE',  ( 31.13667355107491019, -275.5474503757438356, -245.0076206895940061 ) ) ;
#88187=CARTESIAN_POINT ( 'NONE',  ( 37.76200922093805445, -292.2767734184265009, -254.7749289271553721 ) ) ;
#88188=CARTESIAN_POINT ( 'NONE',  ( 37.88321771028709861, -282.0029843431165659, -254.3443301455328651 ) ) ;
#88189=CARTESIAN_POINT ( 'NONE',  ( 22.32098383612148496, -282.4293201077407502, -222.7685966366165928 ) ) ;
#88190=CARTESIAN_POINT ( 'NONE',  ( -102.8978494873622935, -284.3579021650200502, -310.7112799730288657 ) ) ;
#88191=CARTESIAN_POINT ( 'NONE',  ( 7.151849590232073339, -281.0104430209759698, -212.3971315885685840 ) ) ;
#88192=CARTESIAN_POINT ( 'NONE',  ( 35.77081079830085031, -273.2666405000204009, -287.0812184334320705 ) ) ;
#88193=CARTESIAN_POINT ( 'NONE',  ( -109.8947478827530375, -267.1952134479645338, -307.0630218189940024 ) ) ;
#88195=CARTESIAN_POINT ( 'NONE',  ( -62.37982150143177051, -279.3786325072121031, -340.9365589617439127 ) ) ;
#88196=CARTESIAN_POINT ( 'NONE',  ( -90.89323871145485612, -229.7990343503469433, -347.2845633163808543 ) ) ;
#88198=CARTESIAN_POINT ( 'NONE',  ( -75.25642810133714988, -296.8812112239102134, -207.8015043505610322 ) ) ;
#88199=CARTESIAN_POINT ( 'NONE',  ( 24.76848499883414689, -292.4564789224114065, -224.9534996033449090 ) ) ;
#88200=CARTESIAN_POINT ( 'NONE',  ( -21.04059066054967531, -109.3119883923508127, -359.1154128302432582 ) ) ;
#88201=EDGE_CURVE ( 'NONE', #47196, #38497, #17977, .T. ) ;
#88202=CARTESIAN_POINT ( 'NONE',  ( -35.47146142439535765, -296.6498690183287863, -193.9507853632559886 ) ) ;
#88203=CARTESIAN_POINT ( 'NONE',  ( -64.13008383981188842, -287.8072636360128627, -339.1823409630512174 ) ) ;
#88204=CARTESIAN_POINT ( 'NONE',  ( -61.39129890479637908, -297.2281266454388629, -340.6472254639340917 ) ) ;
#88206=CARTESIAN_POINT ( 'NONE',  ( -33.22768840996732820, -287.4200752050302867, -196.9330459988719610 ) ) ;
#88208=CARTESIAN_POINT ( 'NONE',  ( 13.24979206168188739, -295.3064766873507665, -328.1665279788851421 ) ) ;
#88209=CARTESIAN_POINT ( 'NONE',  ( -4.572576537063657298, -286.9884061336192644, -205.0604826033140569 ) ) ;
#88210=CARTESIAN_POINT ( 'NONE',  ( 30.36740316544978313, -297.6770476619486772, -193.7716728435736115 ) ) ;
#88212=CARTESIAN_POINT ( 'NONE',  ( 17.36743678325598950, -293.6117195791124459, -216.3318816005890426 ) ) ;
#88213=CARTESIAN_POINT ( 'NONE',  ( 24.76107106019305704, -293.4410141854605740, -224.9433602868196260 ) ) ;
#88214=CARTESIAN_POINT ( 'NONE',  ( -105.7113890414355666, -291.0618688374010503, -244.6327995941137488 ) ) ;
#88217=CARTESIAN_POINT ( 'NONE',  ( -94.02277199248693762, -275.1617008243414944, -220.3954268340792453 ) ) ;
#88218=CARTESIAN_POINT ( 'NONE',  ( 38.53300312435957409, -274.2146111393961974, -259.8236550624438337 ) ) ;
#88220=CARTESIAN_POINT ( 'NONE',  ( -1.501958393290475868, -276.0975271653778691, -338.4422447049026346 ) ) ;
#88221=CARTESIAN_POINT ( 'NONE',  ( -37.80765668215608599, -296.5260879245860224, -196.6692552082457723 ) ) ;
#88222=CARTESIAN_POINT ( 'NONE',  ( -90.37227467274794890, -281.1526252709547293, -218.3399634613344062 ) ) ;
#88223=CARTESIAN_POINT ( 'NONE',  ( 25.00918386538674554, -274.2413560981182172, -310.7452179939623989 ) ) ;
#88224=CARTESIAN_POINT ( 'NONE',  ( -104.6690256188526433, -274.0214637798055151, -241.2279811572928452 ) ) ;
#88225=CARTESIAN_POINT ( 'NONE',  ( -99.48645739836602786, -274.0264841938550830, -231.6127297359945487 ) ) ;
#88226=CARTESIAN_POINT ( 'NONE',  ( -103.3603874442145667, -274.8086417971169340, -232.6322462306227692 ) ) ;
#88227=CARTESIAN_POINT ( 'NONE',  ( -2.049027641403455391, -272.5372473450477173, -203.7815860377621675 ) ) ;
#88228=CARTESIAN_POINT ( 'NONE',  ( -80.20785339970126415, -296.3015626653618142, -329.5758591503414436 ) ) ;
#88229=CARTESIAN_POINT ( 'NONE',  ( 36.29751644544722211, -292.1323700913396237, -270.7812561167751824 ) ) ;
#88231=CARTESIAN_POINT ( 'NONE',  ( 8.209680046817211974, -276.9402793762799320, -332.4319108869291313 ) ) ;
#88232=CARTESIAN_POINT ( 'NONE',  ( 7.329238533290764579, -274.8475358915682705, -212.6245849761958766 ) ) ;
#88233=CARTESIAN_POINT ( 'NONE',  ( -111.2404638142247961, -283.4888356708507331, -250.3563378992984667 ) ) ;
#88234=CARTESIAN_POINT ( 'NONE',  ( -109.0431402898783375, -298.2614116146913830, -292.9636715070546416 ) ) ;
#88237=CARTESIAN_POINT ( 'NONE',  ( -74.79400943084030473, -284.7368200349844756, -207.5126792201695309 ) ) ;
#88238=CARTESIAN_POINT ( 'NONE',  ( -67.17764200168213051, -281.4422543912177730, -339.3527479199831873 ) ) ;
#88239=CARTESIAN_POINT ( 'NONE',  ( -76.91632690004914252, -275.8295661552189699, -332.9659714203622798 ) ) ;
#88240=CARTESIAN_POINT ( 'NONE',  ( -37.83175530948163612, -275.6330981550337924, -343.9612703428771852 ) ) ;
#88241=CARTESIAN_POINT ( 'NONE',  ( -75.70218864341489962, -281.5404255335116659, -205.8988260176669485 ) ) ;
#88242=CARTESIAN_POINT ( 'NONE',  ( 32.43453334276953370, -276.4547975907180444, -247.4291587977991469 ) ) ;
#88244=CARTESIAN_POINT ( 'NONE',  ( 17.52784463452914565, -273.2197997895094659, -217.4102774602705210 ) ) ;
#88246=CARTESIAN_POINT ( 'NONE',  ( -14.80236189110495992, -282.3435414651202109, -198.5987684119311041 ) ) ;
#88248=CARTESIAN_POINT ( 'NONE',  ( -29.63459085964426265, -288.0691856621139664, -195.1952037397211939 ) ) ;
#88249=AXIS2_PLACEMENT_3D ( 'NONE', #68229, #9985, #30856 ) ;
#88251=CARTESIAN_POINT ( 'NONE',  ( -100.6896029239377839, -288.0107624497654797, -310.6061220982144278 ) ) ;
#88253=CARTESIAN_POINT ( 'NONE',  ( -110.3739708836756108, -271.3446501961809645, -262.1433989632457724 ) ) ;
#88254=CARTESIAN_POINT ( 'NONE',  ( -91.64688067914313763, -289.4076309777720439, -219.7279759228227078 ) ) ;
#88255=CARTESIAN_POINT ( 'NONE',  ( -92.83893396777953910, -239.1568807800618686, -338.3566629249717153 ) ) ;
#88257=CARTESIAN_POINT ( 'NONE',  ( 5.154996196520969853, -286.9685562595444139, -333.7388629163718861 ) ) ;
#88258=CARTESIAN_POINT ( 'NONE',  ( -98.51493802057321147, -283.3998819051982423, -225.1989825478488285 ) ) ;
#88259=CARTESIAN_POINT ( 'NONE',  ( -62.80072885097423807, -291.7112716084420754, -201.9444690110785530 ) ) ;
#88262=CARTESIAN_POINT ( 'NONE',  ( 33.67749910263282942, -282.7242310013076008, -251.0347712590880747 ) ) ;
#88263=CARTESIAN_POINT ( 'NONE',  ( -26.70922734010413180, -283.7164235165128048, -342.7972835085058136 ) ) ;
#88264=CARTESIAN_POINT ( 'NONE',  ( -10.13318631859390706, -290.6785981404049153, -340.6327593413762997 ) ) ;
#88265=CARTESIAN_POINT ( 'NONE',  ( -108.0597576528298731, -273.2744170289830095, -239.8174048061563894 ) ) ;
#88267=CARTESIAN_POINT ( 'NONE',  ( -62.31130467539001927, -287.4541316290829513, -341.7314815628662359 ) ) ;
#88268=CARTESIAN_POINT ( 'NONE',  ( 28.50254742679922515, -275.0299209542463927, -230.3400805502313915 ) ) ;
#88269=CARTESIAN_POINT ( 'NONE',  ( -65.98082745313099906, -293.6554764907412505, -201.4151042775787630 ) ) ;
#88271=CARTESIAN_POINT ( 'NONE',  ( 31.98288692825981272, -278.4805209788417528, -303.7098442033569654 ) ) ;
#88272=CARTESIAN_POINT ( 'NONE',  ( -90.06178684402692625, -275.7943570001564808, -324.0122077690716083 ) ) ;
#88274=CARTESIAN_POINT ( 'NONE',  ( -70.36372970944867689, -296.0240052075956214, -201.6880811971482501 ) ) ;
#88275=CARTESIAN_POINT ( 'NONE',  ( 20.76760079737980647, -274.2776399992562233, -225.9873618624560550 ) ) ;
#88276=CARTESIAN_POINT ( 'NONE',  ( -84.28544903622223217, -292.9126491713624318, -213.5544969866777478 ) ) ;
#88278=CARTESIAN_POINT ( 'NONE',  ( -55.08091300432091941, -292.7596190403543801, -199.3067108432525743 ) ) ;
#88279=CARTESIAN_POINT ( 'NONE',  ( -82.10906341364054128, -287.1921819900448440, -211.4216813088281697 ) ) ;
#88280=CARTESIAN_POINT ( 'NONE',  ( 32.77644349308054217, -294.5874783100049399, -239.9958050992020162 ) ) ;
#88281=CARTESIAN_POINT ( 'NONE',  ( 22.79450742641722272, -295.5040708867605304, -317.6783876256492931 ) ) ;
#88282=CARTESIAN_POINT ( 'NONE',  ( 33.77494002578152532, -293.6034601427674033, -286.8911158114495947 ) ) ;
#88283=CARTESIAN_POINT ( 'NONE',  ( 36.49503310685380342, -289.7212613075241734, -283.5192894324907797 ) ) ;
#88284=CARTESIAN_POINT ( 'NONE',  ( 37.98422382833608424, -281.5183296025614936, -254.3291661651592790 ) ) ;
#88285=CARTESIAN_POINT ( 'NONE',  ( 18.09568570091506245, -296.8208154810340034, -194.8190760047378944 ) ) ;
#88286=CARTESIAN_POINT ( 'NONE',  ( -112.3592484580582038, -284.6025850455986870, -253.0011799902360110 ) ) ;
#88287=CARTESIAN_POINT ( 'NONE',  ( 16.80804729660922447, -278.2562762511470851, -321.7386583726605522 ) ) ;
#88288=CARTESIAN_POINT ( 'NONE',  ( -109.3721152509106815, -283.1621050999826252, -284.4589831772510706 ) ) ;
#88289=CARTESIAN_POINT ( 'NONE',  ( 17.17313334427597482, -286.2742332373839531, -321.8696957180593472 ) ) ;
#88290=CARTESIAN_POINT ( 'NONE',  ( -50.69822842785222150, -278.0228707726343487, -195.7829131917748384 ) ) ;
#88291=CARTESIAN_POINT ( 'NONE',  ( -113.2098679957031493, -271.2709011634024137, -296.4525692007673570 ) ) ;
#88292=CARTESIAN_POINT ( 'NONE',  ( -108.0866798844073884, -284.3005441183248649, -252.1090966943046965 ) ) ;
#88293=CARTESIAN_POINT ( 'NONE',  ( 39.22341567150652963, -282.7874802799650524, -272.7677255736381312 ) ) ;
#88294=CARTESIAN_POINT ( 'NONE',  ( -17.79583782615364385, -287.8647894742294397, -344.5957425130280285 ) ) ;
#88295=CARTESIAN_POINT ( 'NONE',  ( -73.69704314321123206, -279.1265534951251084, -337.3440848844318225 ) ) ;
#88296=CARTESIAN_POINT ( 'NONE',  ( -67.49870513076889722, -278.7547398457653571, -340.6736582788987562 ) ) ;
#88297=CARTESIAN_POINT ( 'NONE',  ( -81.28618619858487193, -279.2693462062475760, -212.0062902534424722 ) ) ;
#88298=CARTESIAN_POINT ( 'NONE',  ( -24.33404948908517795, -276.1987813615330651, -196.8056639094921820 ) ) ;
#88299=CARTESIAN_POINT ( 'NONE',  ( 37.27791870291623866, -285.6330496396946046, -276.6603946458873224 ) ) ;
#88300=CARTESIAN_POINT ( 'NONE',  ( -70.27467607839722064, -291.0789694156782161, -339.0912397889829890 ) ) ;
#88301=CARTESIAN_POINT ( 'NONE',  ( -5.419282164645363942, -293.5423160424007278, -336.3688133059591792 ) ) ;
#88303=CARTESIAN_POINT ( 'NONE',  ( -45.09719836104773094, -294.8196469527659929, -343.0197338190831147 ) ) ;
#88304=CARTESIAN_POINT ( 'NONE',  ( -111.6191986383296495, -291.3913850031715924, -289.5014578736276576 ) ) ;
#88305=CARTESIAN_POINT ( 'NONE',  ( -38.36360349920153112, -280.6904267470862919, -197.2539093970831914 ) ) ;
#88306=CARTESIAN_POINT ( 'NONE',  ( 75.83355947227427407, -298.3581913397087533, -193.6903554288949749 ) ) ;
#88307=CARTESIAN_POINT ( 'NONE',  ( 19.55442187814812272, -288.9077138713660702, -322.1121951704050730 ) ) ;
#88308=CARTESIAN_POINT ( 'NONE',  ( -62.75266672728255202, -289.7072037028835894, -343.0812803795569721 ) ) ;
#88309=CARTESIAN_POINT ( 'NONE',  ( -73.56980829239275010, -285.8904698062691523, -206.9462098343767593 ) ) ;
#88310=CARTESIAN_POINT ( 'NONE',  ( 64.47034098757669085, 48.08436262820399776, -318.7852478018613169 ) ) ;
#88312=CARTESIAN_POINT ( 'NONE',  ( 23.85667543695174686, -22.61630356684642962, -343.2597395675320513 ) ) ;
#88313=CARTESIAN_POINT ( 'NONE',  ( -39.01470583219347077, -140.0999525806348345, -360.8708370586243177 ) ) ;
#88314=CARTESIAN_POINT ( 'NONE',  ( -32.41988592551756199, -276.1858179835649025, -343.4069310343268739 ) ) ;
#88315=CARTESIAN_POINT ( 'NONE',  ( -64.46022434401164958, -276.3348179571497099, -338.5238552467184832 ) ) ;
#88316=CARTESIAN_POINT ( 'NONE',  ( -110.0804957009435014, -272.5366084470006740, -245.1656439823766505 ) ) ;
#88317=CARTESIAN_POINT ( 'NONE',  ( -11.02755183398383210, -93.07797461907387060, -357.3970400885787058 ) ) ;
#88319=CARTESIAN_POINT ( 'NONE',  ( -41.37530129399917200, -275.7867418359247722, -346.7746893807156425 ) ) ;
#88320=AXIS2_PLACEMENT_3D ( 'NONE', #22245, #42129, #42605 ) ;
#88321=CARTESIAN_POINT ( 'NONE',  ( -36.26601005852802473, -296.7990116537307586, -346.3531046861765503 ) ) ;
#88323=CARTESIAN_POINT ( 'NONE',  ( -81.77143365266174158, -291.9209641106515392, -212.2972044397519369 ) ) ;
#88324=CARTESIAN_POINT ( 'NONE',  ( 7.860778187331947109, -299.4074188288229834, -193.5166010588536096 ) ) ;
#88325=CARTESIAN_POINT ( 'NONE',  ( 14.41890826709834172, -286.9900973570545943, -322.5347022575787150 ) ) ;
#88326=CARTESIAN_POINT ( 'NONE',  ( -34.76829161298174853, -298.5759069919729427, -193.4224475131729548 ) ) ;
#88327=CARTESIAN_POINT ( 'NONE',  ( -102.7672165908978172, -296.2785247921804057, -302.8559199959760804 ) ) ;
#88331=CARTESIAN_POINT ( 'NONE',  ( -69.37457967765314493, -281.5541621010550557, -201.9130218495632789 ) ) ;
#88332=CARTESIAN_POINT ( 'NONE',  ( 25.87618300709601726, -281.6398420643884037, -314.2366081631833481 ) ) ;
#88334=CARTESIAN_POINT ( 'NONE',  ( -105.8078928284799218, -279.9819793890968640, -244.0156876919396609 ) ) ;
#88335=CARTESIAN_POINT ( 'NONE',  ( -96.25434435633232511, -279.6594397931527283, -318.3739276372007225 ) ) ;
#88336=CARTESIAN_POINT ( 'NONE',  ( -29.90079146808069765, -272.6279161110299469, -197.0444034459961529 ) ) ;
#88339=CARTESIAN_POINT ( 'NONE',  ( 15.25790792428147746, -280.9872562388425195, -219.6699268078835132 ) ) ;
#88340=CARTESIAN_POINT ( 'NONE',  ( 16.84861157140450061, -277.1073962702839140, -324.9108227841372241 ) ) ;
#88342=CARTESIAN_POINT ( 'NONE',  ( 17.45970322547478304, -278.2692377983377696, -321.5647002748431191 ) ) ;
#88343=CARTESIAN_POINT ( 'NONE',  ( -111.2620745014318118, -276.8822345962194618, -289.7615970377026429 ) ) ;
#88345=CARTESIAN_POINT ( 'NONE',  ( 82.64890176555634582, -299.5541904835141622, -195.3611179825600175 ) ) ;
#88346=CARTESIAN_POINT ( 'NONE',  ( 37.97662328196414450, -283.5621720336718568, -272.7184381945962173 ) ) ;
#88347=CARTESIAN_POINT ( 'NONE',  ( -104.8481244732191584, -290.1283952248891183, -242.0249942809589072 ) ) ;
#88348=CARTESIAN_POINT ( 'NONE',  ( -12.72847449836845257, -285.7125162726246685, -197.5085139762025221 ) ) ;
#88349=CARTESIAN_POINT ( 'NONE',  ( -53.93840260113621099, -281.5078336105353856, -342.5424498482227591 ) ) ;
#88350=CARTESIAN_POINT ( 'NONE',  ( -23.97614164480430077, -281.4527915258097437, -342.7264187973819958 ) ) ;
#88351=CARTESIAN_POINT ( 'NONE',  ( 33.21308620789464783, -285.3228047815757691, -246.6264108556927681 ) ) ;
#88352=CARTESIAN_POINT ( 'NONE',  ( 34.14364879179218804, -282.5388704208897934, -253.7185401766971609 ) ) ;
#88353=CARTESIAN_POINT ( 'NONE',  ( -97.93575550138670849, -271.1552731541447088, -226.0781938378329983 ) ) ;
#88354=CARTESIAN_POINT ( 'NONE',  ( 23.60288138149907056, -280.5672334012831470, -316.1016733135513732 ) ) ;
#88355=CARTESIAN_POINT ( 'NONE',  ( 34.36708847235066600, -295.2690317615726485, -248.3872633632298346 ) ) ;
#88357=CARTESIAN_POINT ( 'NONE',  ( -10.66892226079047212, -288.3992486794542174, -200.0305657835561703 ) ) ;
#88359=CARTESIAN_POINT ( 'NONE',  ( -81.11641203582675530, -293.3826606780352222, -208.7730607559209659 ) ) ;
#88360=CARTESIAN_POINT ( 'NONE',  ( 36.82311238471707782, -273.4075654045568058, -259.1129180082863854 ) ) ;
#88361=CARTESIAN_POINT ( 'NONE',  ( 31.53812641407240136, -287.1892287272665385, -304.5358678678690012 ) ) ;
#88362=CARTESIAN_POINT ( 'NONE',  ( 33.40174502640356735, -291.6747861610853079, -249.1656847508699570 ) ) ;
#88364=CARTESIAN_POINT ( 'NONE',  ( -108.7650005277292138, -277.4639510712643755, -253.0418905301113455 ) ) ;
#88365=CARTESIAN_POINT ( 'NONE',  ( -90.92123764730045821, -295.4216403587806212, -218.9056892819436086 ) ) ;
#88366=CARTESIAN_POINT ( 'NONE',  ( -76.11479323089244531, -290.8973399789280734, -332.7942079984620136 ) ) ;
#88369=CARTESIAN_POINT ( 'NONE',  ( 37.91921114877387566, -292.1919155545822946, -283.0299677060057206 ) ) ;
#88370=CARTESIAN_POINT ( 'NONE',  ( 34.77345160926238066, -288.9476863410220062, -254.6816630359113844 ) ) ;
#88371=CARTESIAN_POINT ( 'NONE',  ( -110.9461476636871708, -288.5520315873618529, -289.2907138257573365 ) ) ;
#88372=CARTESIAN_POINT ( 'NONE',  ( 36.04098063235412752, -289.0579307670378171, -276.5126682850371367 ) ) ;
#88374=CARTESIAN_POINT ( 'NONE',  ( 13.24383515989090654, -287.5840732446478683, -217.4357199264438236 ) ) ;
#88375=CARTESIAN_POINT ( 'NONE',  ( -36.27195443380546180, -297.0187270494103018, -345.7215522481367884 ) ) ;
#88377=CARTESIAN_POINT ( 'NONE',  ( -77.91302123592927842, -290.7890664145993469, -335.3997267615584406 ) ) ;
#88378=CARTESIAN_POINT ( 'NONE',  ( -20.10736608977926920, -278.2925059415758824, -196.9495921673949113 ) ) ;
#88379=CARTESIAN_POINT ( 'NONE',  ( -70.28811465792983881, -277.8077659595787168, -339.9476580797378915 ) ) ;
#88380=CARTESIAN_POINT ( 'NONE',  ( -74.99388626688092074, -279.2314462878293284, -203.2190509119599540 ) ) ;
#88381=CARTESIAN_POINT ( 'NONE',  ( -78.43811258538219988, -299.4764012231978541, -207.9858187344139537 ) ) ;
#88382=CARTESIAN_POINT ( 'NONE',  ( -104.0047476339076411, -283.0067381606190793, -235.9948737452589285 ) ) ;
#88383=CARTESIAN_POINT ( 'NONE',  ( -110.5111785248877254, -273.3798195326398286, -270.3716561707263963 ) ) ;
#88384=CARTESIAN_POINT ( 'NONE',  ( 16.16586465980358511, -278.9604871399368449, -218.8308210222380126 ) ) ;
#88385=CARTESIAN_POINT ( 'NONE',  ( -84.85552501192522357, -281.7072597161362637, -328.3907405089061058 ) ) ;
#88387=CARTESIAN_POINT ( 'NONE',  ( 27.05323622525508043, -274.5746043185469034, -311.3982767116811488 ) ) ;
#88388=CARTESIAN_POINT ( 'NONE',  ( -34.46516265151763037, -299.6089241566747319, -196.6670189504422694 ) ) ;
#88389=CARTESIAN_POINT ( 'NONE',  ( -111.5792251037152027, -283.2300863215691038, -289.6559415013193757 ) ) ;
#88390=CARTESIAN_POINT ( 'NONE',  ( -84.23466017814951101, -298.3302029245483595, -214.0413749894937894 ) ) ;
#88391=CARTESIAN_POINT ( 'NONE',  ( -110.4784897142456401, -274.2593736009206964, -248.0528316499418224 ) ) ;
#88392=CARTESIAN_POINT ( 'NONE',  ( 15.61029072797740547, -275.9434760508664226, -320.6420701529017379 ) ) ;
#88393=CARTESIAN_POINT ( 'NONE',  ( 35.58670770306607523, -295.3268785512871659, -252.8006764312624739 ) ) ;
#88394=CARTESIAN_POINT ( 'NONE',  ( 7.936226338078881781, -288.6194067191822796, -332.7077613498963160 ) ) ;
#88396=CARTESIAN_POINT ( 'NONE',  ( -74.28218145964285668, -277.6448296314165987, -204.4466655615579214 ) ) ;
#88398=CARTESIAN_POINT ( 'NONE',  ( -112.8684122999209620, -290.1971598758132700, -285.4184812480793880 ) ) ;
#88399=CARTESIAN_POINT ( 'NONE',  ( -39.97852786529680458, -288.1447092853567824, -343.5986674098405729 ) ) ;
#88400=CARTESIAN_POINT ( 'NONE',  ( 26.36727644629094414, -291.0193906694595967, -230.6881069424669306 ) ) ;
#88403=CARTESIAN_POINT ( 'NONE',  ( -93.48310235590990658, -290.7228100030895348, -223.5855052179659879 ) ) ;
#88405=CARTESIAN_POINT ( 'NONE',  ( -75.99863040647869639, -286.4906103935792316, -203.9789989813614568 ) ) ;
#88406=CARTESIAN_POINT ( 'NONE',  ( 34.45848030099739390, -290.0519495502701943, -270.3284710469131937 ) ) ;
#88407=CARTESIAN_POINT ( 'NONE',  ( 35.25995479463410476, -292.9279873997329560, -295.4602537846284918 ) ) ;
#88408=CARTESIAN_POINT ( 'NONE',  ( 1.855952159964453507, -283.8543508477170576, -336.0637992646063026 ) ) ;
#88409=CARTESIAN_POINT ( 'NONE',  ( -89.66137462613536968, -285.1223172450450534, -219.3803136969849561 ) ) ;
#88410=CARTESIAN_POINT ( 'NONE',  ( 34.06967216978969049, -277.0955781586472426, -287.7825261683270242 ) ) ;
#88411=CARTESIAN_POINT ( 'NONE',  ( -27.87326942609925950, -290.1929268393409416, -196.2673747515878802 ) ) ;
#88413=CARTESIAN_POINT ( 'NONE',  ( 17.59289884355095168, -273.6546396988354672, -221.6101244988556971 ) ) ;
#88415=CARTESIAN_POINT ( 'NONE',  ( 24.80950920047307307, -22.49099280560490399, -345.4124233396505019 ) ) ;
#88416=CARTESIAN_POINT ( 'NONE',  ( 38.79500651294415547, -293.3609267962822855, -281.7165657227873226 ) ) ;
#88417=CARTESIAN_POINT ( 'NONE',  ( -80.15712208741508960, -287.3880858171455088, -209.4032094800290906 ) ) ;
#88418=CARTESIAN_POINT ( 'NONE',  ( -93.45388892569485506, -296.9161152799579213, -322.6577427359322314 ) ) ;
#88419=CARTESIAN_POINT ( 'NONE',  ( 35.78209718498725778, -288.1764353590843939, -268.3013227700150765 ) ) ;
#88421=CARTESIAN_POINT ( 'NONE',  ( -96.87952786620257939, -276.9584842756896137, -318.8385659375060754 ) ) ;
#88422=CARTESIAN_POINT ( 'NONE',  ( 38.74979561751858625, -294.0599818243625805, -258.8956749405239748 ) ) ;
#88423=CARTESIAN_POINT ( 'NONE',  ( 36.52085021038865875, -285.4766479620708992, -253.4325027342885903 ) ) ;
#88424=CARTESIAN_POINT ( 'NONE',  ( -3.234333105599584979, -294.9473619252771073, -339.3860928775064281 ) ) ;
#88425=CARTESIAN_POINT ( 'NONE',  ( -93.45881006288888670, -291.5483048053866355, -223.6194661385467555 ) ) ;
#88426=DIRECTION ( 'NONE',  ( 0.000000000000000000, 0.000000000000000000, -1.000000000000000000 ) ) ;
#88429=CARTESIAN_POINT ( 'NONE',  ( -73.30353221983686751, -287.1046034826480309, -203.0013678776625738 ) ) ;
#88430=CARTESIAN_POINT ( 'NONE',  ( -99.90806341382575795, -275.4094976428775681, -320.2154176792147382 ) ) ;
#88432=CARTESIAN_POINT ( 'NONE',  ( -108.7294473697317869, -283.2527957973595676, -287.0898107364959628 ) ) ;
#88433=CARTESIAN_POINT ( 'NONE',  ( -110.5282576224401936, -278.5210733337091256, -246.3283510950774939 ) ) ;
#88434=CARTESIAN_POINT ( 'NONE',  ( 37.34815239942914644, -283.4927118035662943, -265.7292335484566479 ) ) ;
#88435=CARTESIAN_POINT ( 'NONE',  ( -46.01903522638156829, -156.0925041209123947, -363.9939798654107790 ) ) ;
#88436=CARTESIAN_POINT ( 'NONE',  ( 25.43579381673064077, -280.7070675659978178, -313.9454875174558879 ) ) ;
#88437=CARTESIAN_POINT ( 'NONE',  ( -38.62853349285001769, -284.0560806223729173, -195.7146434152016354 ) ) ;
#88438=CARTESIAN_POINT ( 'NONE',  ( -55.06798076574337841, -275.6869646415621560, -196.6991572936201749 ) ) ;
#88439=CARTESIAN_POINT ( 'NONE',  ( -60.54137627549009437, -298.2354512486919020, -201.0272768415937321 ) ) ;
#88440=CARTESIAN_POINT ( 'NONE',  ( -38.36585319624217760, -293.7500796885653926, -343.8471342714623802 ) ) ;
#88441=CARTESIAN_POINT ( 'NONE',  ( -91.25165161343427656, -278.4455034643027034, -325.2720703117487346 ) ) ;
#88442=CARTESIAN_POINT ( 'NONE',  ( -66.80266182023279953, -277.4492729165524452, -337.1522232000482404 ) ) ;
#88443=CARTESIAN_POINT ( 'NONE',  ( -43.28354042979076866, -298.9202365054322286, -193.7736677831919110 ) ) ;
#88444=CARTESIAN_POINT ( 'NONE',  ( -51.27002410595544291, -276.1465561689792594, -345.7765958375545665 ) ) ;
#88445=CARTESIAN_POINT ( 'NONE',  ( -64.04501568493247987, -182.5871740904552212, -362.3045948284940323 ) ) ;
#88446=CARTESIAN_POINT ( 'NONE',  ( -29.56210322979992000, -274.9535946256202124, -345.0075661269856369 ) ) ;
#88448=CARTESIAN_POINT ( 'NONE',  ( -86.00598603367318162, -297.1368840681679444, -329.2711643973815399 ) ) ;
#88451=CARTESIAN_POINT ( 'NONE',  ( -42.94287154574270460, -284.2040399720792720, -343.5062384627763095 ) ) ;
#88452=CARTESIAN_POINT ( 'NONE',  ( -113.1952159813393735, -286.2450175381646886, -275.6696175899485866 ) ) ;
#88453=CARTESIAN_POINT ( 'NONE',  ( -70.02056274128207747, -284.9585084809592672, -204.9561418139582258 ) ) ;
#88454=CARTESIAN_POINT ( 'NONE',  ( -85.64406883759544087, -276.1331468154814388, -326.2259756062181850 ) ) ;
#88455=CARTESIAN_POINT ( 'NONE',  ( -95.94654224486873773, -287.0440923702187774, -224.7736176087444449 ) ) ;
#88456=CARTESIAN_POINT ( 'NONE',  ( -43.79267295890605993, -278.4491646523954387, -196.8999668992775298 ) ) ;
#88457=CARTESIAN_POINT ( 'NONE',  ( -3.713473766556704803, -277.6771198893313795, -335.5022606361942508 ) ) ;
#88459=CARTESIAN_POINT ( 'NONE',  ( -109.1913906023498413, -273.2227359036598955, -256.8385640283184443 ) ) ;
#88460=CARTESIAN_POINT ( 'NONE',  ( 36.01849478172940877, -282.0672323828374033, -247.5041579204160769 ) ) ;
#88461=CARTESIAN_POINT ( 'NONE',  ( 39.34986729319370369, -281.9674126951711628, -264.2023527192749270 ) ) ;
#88466=CARTESIAN_POINT ( 'NONE',  ( 4.477828423660729307, -288.4698363977563531, -207.1208566238755679 ) ) ;
#88467=CARTESIAN_POINT ( 'NONE',  ( -101.3509117173909857, -296.2325176133599598, -234.9291753567264038 ) ) ;
#88468=CARTESIAN_POINT ( 'NONE',  ( -25.02957679759807874, -291.5538233017906009, -194.4550944704950837 ) ) ;
#88469=CARTESIAN_POINT ( 'NONE',  ( 36.24623652190252443, -285.9692924546910149, -265.5606461922162680 ) ) ;
#88470=CARTESIAN_POINT ( 'NONE',  ( 18.25889362138731542, -286.8091116780663583, -318.6447420614047132 ) ) ;
#88471=CARTESIAN_POINT ( 'NONE',  ( -30.50952235267011403, -287.3454072453388903, -197.2316484089523954 ) ) ;
#88472=CARTESIAN_POINT ( 'NONE',  ( -85.82230911780693816, -275.7228669224093096, -327.6534832507173860 ) ) ;
#88473=CARTESIAN_POINT ( 'NONE',  ( -23.47770371204173401, -287.2777825434094439, -345.3428339857504739 ) ) ;
#88474=CARTESIAN_POINT ( 'NONE',  ( 12.88802453970373740, -288.7529821478595977, -214.5960837472935054 ) ) ;
#88475=CARTESIAN_POINT ( 'NONE',  ( -84.04596688189603526, -287.6916727221295673, -329.3235533382184599 ) ) ;
#88476=CARTESIAN_POINT ( 'NONE',  ( 33.88178482580691053, -282.7182723827438053, -287.4621928760510627 ) ) ;
#88477=CARTESIAN_POINT ( 'NONE',  ( -110.2233965358838788, -292.7886552872353718, -251.9166283540837981 ) ) ;
#88478=CARTESIAN_POINT ( 'NONE',  ( 82.13009088781083733, -301.0284103969703438, -194.0088967232378536 ) ) ;
#88479=DIRECTION ( 'NONE',  ( 0.000000000000000000, 1.000000000000000000, -1.224646799147353207E-16 ) ) ;
#88480=CARTESIAN_POINT ( 'NONE',  ( -70.12677391686942485, -299.5437175786609600, -202.2843000516843119 ) ) ;
#88482=CARTESIAN_POINT ( 'NONE',  ( 21.46485241405459021, -280.1401802729444626, -226.8154255989534249 ) ) ;
#88483=CARTESIAN_POINT ( 'NONE',  ( 14.74183822126638432, -278.7850881649446251, -216.3229377038205996 ) ) ;
#88484=CARTESIAN_POINT ( 'NONE',  ( 22.15509706543970125, -293.4035999149492682, -319.0057344757882447 ) ) ;
#88485=CARTESIAN_POINT ( 'NONE',  ( -63.34244523359843271, -296.1076670961292052, -201.2389648726340283 ) ) ;
#88486=CARTESIAN_POINT ( 'NONE',  ( -9.471482530709096181, -274.7649470605410897, -339.4007788391619442 ) ) ;
#88487=CARTESIAN_POINT ( 'NONE',  ( 6.369606081040358525, -295.7598689177297615, -329.5055550071194830 ) ) ;
#88488=DIRECTION ( 'NONE',  ( 0.000000000000000000, 0.000000000000000000, -1.000000000000000000 ) ) ;
#88489=CARTESIAN_POINT ( 'NONE',  ( -113.7517970869267003, -271.1629708653914008, -267.4974886568448369 ) ) ;
#88490=CARTESIAN_POINT ( 'NONE',  ( -111.6194279198050623, -294.5889328096234294, -286.3858854163530054 ) ) ;
#88491=CARTESIAN_POINT ( 'NONE',  ( -55.17255378784323483, -293.2435614495827849, -198.9647905334667541 ) ) ;
#88492=LINE ( 'NONE', #31219, #15749 ) ;
#88493=CARTESIAN_POINT ( 'NONE',  ( 34.37274956735878106, -294.1644075634281990, -255.8821873482296496 ) ) ;
#88495=CARTESIAN_POINT ( 'NONE',  ( -90.71972796632600478, -283.3198945101642039, -217.1709596275337901 ) ) ;
#88496=CARTESIAN_POINT ( 'NONE',  ( -69.72406891981063382, -295.4908810974197877, -335.7857478358227468 ) ) ;
#88497=CARTESIAN_POINT ( 'NONE',  ( -111.7212154822737062, -284.8037971640941350, -250.2436990138195370 ) ) ;
#88498=CARTESIAN_POINT ( 'NONE',  ( 26.61912792095626301, -282.9343685800570256, -230.0346814948160556 ) ) ;
#88499=CARTESIAN_POINT ( 'NONE',  ( -63.19033816739273846, -285.3911756945738034, -197.8518620009969311 ) ) ;
#88500=CARTESIAN_POINT ( 'NONE',  ( -98.23879439052350904, -289.1458171233265944, -226.7812969986545966 ) ) ;
#88501=CARTESIAN_POINT ( 'NONE',  ( -112.3381139276885108, -270.1608578419545665, -261.8788190812425682 ) ) ;
#88502=CARTESIAN_POINT ( 'NONE',  ( -77.30325992398987012, -284.1891223428384023, -208.6215973698091091 ) ) ;
#88503=CARTESIAN_POINT ( 'NONE',  ( -113.0570721683566546, -289.3193766518436973, -282.5543516298441205 ) ) ;
#88505=CARTESIAN_POINT ( 'NONE',  ( -58.61963103197609115, -296.9320747185212781, -341.0271640727563067 ) ) ;
#88506=CARTESIAN_POINT ( 'NONE',  ( -109.0594940703633000, -280.3149441631099990, -243.8422918023784973 ) ) ;
#88507=CARTESIAN_POINT ( 'NONE',  ( 33.92249740727758933, -291.8895146090274579, -295.0121052964305477 ) ) ;
#88508=CARTESIAN_POINT ( 'NONE',  ( 2.719130064279232872, -280.2722908003071893, -209.2495025191904290 ) ) ;
#88509=CARTESIAN_POINT ( 'NONE',  ( -56.06822933098914064, -295.4535948077426042, -345.0492502961826062 ) ) ;
#88510=CARTESIAN_POINT ( 'NONE',  ( -69.16367997142182844, -283.7167501598232775, -201.8147253816856335 ) ) ;
#88511=CARTESIAN_POINT ( 'NONE',  ( -112.2157321526965745, -280.6081071514298628, -266.0160087148465209 ) ) ;
#88512=CARTESIAN_POINT ( 'NONE',  ( -45.12762775168771157, -294.2117741372102842, -343.2320005252281021 ) ) ;
#88513=CARTESIAN_POINT ( 'NONE',  ( -23.78527057963961866, -296.2216931636220920, -195.3657311741189631 ) ) ;
#88514=EDGE_LOOP ( 'NONE', ( #9939, #76068, #4782, #14204 ) ) ;
#88515=CARTESIAN_POINT ( 'NONE',  ( 82.64890176555634582, -299.5541904835138780, -192.9651424135223863 ) ) ;
#88516=CARTESIAN_POINT ( 'NONE',  ( -8.637638259825131115, -282.4095485859864425, -201.4559393924883466 ) ) ;
#88517=CARTESIAN_POINT ( 'NONE',  ( -108.5355912949711694, -296.2761499308048201, -253.9471512955446713 ) ) ;
#88519=CARTESIAN_POINT ( 'NONE',  ( -20.25526795762938548, -274.3380690714490697, -345.3683826091709648 ) ) ;
#88520=CARTESIAN_POINT ( 'NONE',  ( -10.39464456842249618, -273.5920247200083963, -198.3460847391739605 ) ) ;
#88521=CARTESIAN_POINT ( 'NONE',  ( 0.4901084896368336219, -289.8745069564153596, -336.9195063054415300 ) ) ;
#88522=CARTESIAN_POINT ( 'NONE',  ( -108.6631783807477944, -290.1794428326551838, -285.9835141821380944 ) ) ;
#88523=CARTESIAN_POINT ( 'NONE',  ( -46.56222053103841318, -281.4532781753128461, -197.1953051579458531 ) ) ;
#88524=CARTESIAN_POINT ( 'NONE',  ( 14.03918459206960456, -276.3883281344809575, -217.3852263004769156 ) ) ;
#88525=CARTESIAN_POINT ( 'NONE',  ( -43.77065947555172443, -278.7641600716794414, -197.1956397570254467 ) ) ;
#88526=CARTESIAN_POINT ( 'NONE',  ( 28.53534170143589677, -278.0298666276397057, -306.3196615243484189 ) ) ;
#88528=CARTESIAN_POINT ( 'NONE',  ( -73.94299285587297277, -273.4134409584095806, -202.5571389455984956 ) ) ;
#88529=CARTESIAN_POINT ( 'NONE',  ( -9.205429504363960902, -294.3429056573678508, -201.3884716815977356 ) ) ;
#88533=CARTESIAN_POINT ( 'NONE',  ( 16.62666955183015105, -290.9489003618078868, -217.1109015138176233 ) ) ;
#88534=CARTESIAN_POINT ( 'NONE',  ( -100.7680774266537753, -272.5575023856835628, -233.9953221529800658 ) ) ;
#88536=CARTESIAN_POINT ( 'NONE',  ( 24.24333332018625242, -294.4686228622493331, -225.3056920149629434 ) ) ;
#88537=CARTESIAN_POINT ( 'NONE',  ( -37.37352853689063181, -300.5519495502701375, -190.3611179825600175 ) ) ;
#88538=CARTESIAN_POINT ( 'NONE',  ( -24.86050574439200744, -288.2117554192093394, -196.5233848264242340 ) ) ;
#88539=CARTESIAN_POINT ( 'NONE',  ( 23.95320766709258820, -274.1370893526035388, -313.3797822893422449 ) ) ;
#88540=CARTESIAN_POINT ( 'NONE',  ( 16.47118851754191482, -276.7439802151927211, -218.8522281758815780 ) ) ;
#88541=CARTESIAN_POINT ( 'NONE',  ( -67.11806428619449605, -289.7385636203684385, -202.1358855703558675 ) ) ;
#88542=CARTESIAN_POINT ( 'NONE',  ( -36.78579942146701853, -281.9194800908829279, -194.5855178512138650 ) ) ;
#88545=CARTESIAN_POINT ( 'NONE',  ( -71.46380203444815038, -282.8640336087179321, -335.0107493035188782 ) ) ;
#88546=CARTESIAN_POINT ( 'NONE',  ( -103.3327688262298665, -279.1195643356890059, -309.5378694227637766 ) ) ;
#88547=CARTESIAN_POINT ( 'NONE',  ( -69.03624981959376328, -282.2546929003748346, -340.1140013045026080 ) ) ;
#88548=CARTESIAN_POINT ( 'NONE',  ( -73.97398428856054409, -278.4677835439621845, -337.8364018855518793 ) ) ;
#88550=CARTESIAN_POINT ( 'NONE',  ( 21.21116831999255581, -277.7366993535750908, -319.2923896937128347 ) ) ;
#88551=CARTESIAN_POINT ( 'NONE',  ( -82.13390479932378696, -287.9090924074130839, -214.2458315076590907 ) ) ;
#88553=CARTESIAN_POINT ( 'NONE',  ( -100.4014615540004627, -298.0042605503799109, -311.0575292080845884 ) ) ;
#88554=CARTESIAN_POINT ( 'NONE',  ( -109.9270766119712164, -291.4956652911773745, -280.7267191666221606 ) ) ;
#88555=CARTESIAN_POINT ( 'NONE',  ( -69.99315480742112072, -275.5044141797649218, -337.4999981691831294 ) ) ;
#88556=CARTESIAN_POINT ( 'NONE',  ( -26.26977446216316281, -290.6732074012569456, -345.5368219965002936 ) ) ;
#88557=CARTESIAN_POINT ( 'NONE',  ( -96.83949755286823802, -290.4943465611121383, -227.8031088026038731 ) ) ;
#88558=CARTESIAN_POINT ( 'NONE',  ( 33.98292406371783869, -287.4279761727746632, -299.3530377534742115 ) ) ;
#88560=CARTESIAN_POINT ( 'NONE',  ( -104.8532600564601722, -282.5552102055612522, -300.1710104541108990 ) ) ;
#88561=CARTESIAN_POINT ( 'NONE',  ( -61.63727555923826174, -291.2316389326693979, -340.5080387541444793 ) ) ;
#88562=CARTESIAN_POINT ( 'NONE',  ( -97.12606839542758053, -283.6291752243014912, -227.2520467831803614 ) ) ;
#88563=CARTESIAN_POINT ( 'NONE',  ( -2.932933465215186164, -281.8320255687440863, -205.4062556964880741 ) ) ;
#88564=CARTESIAN_POINT ( 'NONE',  ( 21.31699990451652482, -289.1625275061616662, -319.8785606080607522 ) ) ;
#88565=CARTESIAN_POINT ( 'NONE',  ( -105.3227668628072564, -278.6868174819926480, -297.1298125180252896 ) ) ;
#88566=CARTESIAN_POINT ( 'NONE',  ( 27.72324783100738443, -291.8143472972927270, -229.8311499959664843 ) ) ;
#88567=CARTESIAN_POINT ( 'NONE',  ( -33.74513533688882205, -286.8991606241152681, -193.6068116376738431 ) ) ;
#88568=CARTESIAN_POINT ( 'NONE',  ( 39.54315984231079284, -288.0952187408752820, -274.4134374820295648 ) ) ;
#88569=CARTESIAN_POINT ( 'NONE',  ( -51.01581621922784393, -283.3983365598688806, -342.1205637136178552 ) ) ;
#88572=CARTESIAN_POINT ( 'NONE',  ( 36.21693448439535246, -295.1818018899278968, -252.2108353981194000 ) ) ;
#88573=CARTESIAN_POINT ( 'NONE',  ( 36.61553010370923289, -292.4837718926271464, -289.9475002516084601 ) ) ;
#88574=CARTESIAN_POINT ( 'NONE',  ( 25.57159628898023129, -275.1246497180182473, -307.8487903784329660 ) ) ;
#88575=CARTESIAN_POINT ( 'NONE',  ( -62.80346509521832132, -297.0777911781560761, -197.8007203044634537 ) ) ;
#88576=CARTESIAN_POINT ( 'NONE',  ( -2.090914190285290353, -291.0076424977363558, -205.6313333339709288 ) ) ;
#88577=CARTESIAN_POINT ( 'NONE',  ( -92.58653704136588658, -295.4867382466309209, -221.1068591912486454 ) ) ;
#88578=CARTESIAN_POINT ( 'NONE',  ( -90.11241298346455153, -292.4903711764793570, -219.3475671408286019 ) ) ;
#88579=CARTESIAN_POINT ( 'NONE',  ( 21.58309136429705433, -295.2407226535077598, -313.9741323465929099 ) ) ;
#88581=CARTESIAN_POINT ( 'NONE',  ( -2.832400743315037328, -292.5968778718313956, -337.1378855418639660 ) ) ;
#88582=CARTESIAN_POINT ( 'NONE',  ( -109.7411779152843962, -298.8045916485828002, -250.7344950078710895 ) ) ;
#88583=CARTESIAN_POINT ( 'NONE',  ( 34.79706119545801357, -288.3236311210037570, -257.4496525727625453 ) ) ;
#88584=CARTESIAN_POINT ( 'NONE',  ( 31.52699331031440266, -277.9309207650316580, -300.9472237163761292 ) ) ;
#88585=CARTESIAN_POINT ( 'NONE',  ( -113.7175655017542653, -277.2933064376213679, -265.8861364156356899 ) ) ;
#88586=CARTESIAN_POINT ( 'NONE',  ( -10.37557693812024873, -273.7434196691516490, -198.2896006618775004 ) ) ;
#88587=CARTESIAN_POINT ( 'NONE',  ( 36.56650901000911347, -279.7523137793989463, -279.6619491718978452 ) ) ;
#88588=CARTESIAN_POINT ( 'NONE',  ( -99.58364084687843842, -277.5398315875208937, -226.4022595844365924 ) ) ;
#88589=CARTESIAN_POINT ( 'NONE',  ( -96.00804401660965937, -294.6191045367037873, -314.6481352243256424 ) ) ;
#88591=CARTESIAN_POINT ( 'NONE',  ( -19.25441361073336211, -274.9423732675803080, -199.4796509324681040 ) ) ;
#88593=CARTESIAN_POINT ( 'NONE',  ( -112.5447354075375870, -288.6334258410384450, -265.5746490239581021 ) ) ;
#88594=CARTESIAN_POINT ( 'NONE',  ( -68.05387736649520036, -289.4444033109572274, -340.9710476615807124 ) ) ;
#88595=CARTESIAN_POINT ( 'NONE',  ( -36.93397297826390258, -300.0371189401193419, -195.0057727177184290 ) ) ;
#88596=CARTESIAN_POINT ( 'NONE',  ( -111.8738659412356071, -294.6454663210720923, -263.0969798992497317 ) ) ;
#88597=CARTESIAN_POINT ( 'NONE',  ( -106.8638966795725196, -283.3292937786462744, -303.0845500557905439 ) ) ;
#88599=CARTESIAN_POINT ( 'NONE',  ( -76.07019371423882603, -281.5689830938668479, -334.6472283539877139 ) ) ;
#88602=CARTESIAN_POINT ( 'NONE',  ( -81.95831902828879834, -290.2238142994540908, -212.0174204110471692 ) ) ;
#88603=CARTESIAN_POINT ( 'NONE',  ( -111.1028298048073850, -282.5773051127588928, -279.1819974564393760 ) ) ;
#88606=CARTESIAN_POINT ( 'NONE',  ( -16.86267289465900276, -290.3163318994787119, -198.1571647211805782 ) ) ;
#88607=CARTESIAN_POINT ( 'NONE',  ( -35.07284752423389307, -278.6233188190329315, -344.1262366008237450 ) ) ;
#88608=CARTESIAN_POINT ( 'NONE',  ( -38.70998809155816645, -284.2740262467856383, -346.9518256965196201 ) ) ;
#88609=CARTESIAN_POINT ( 'NONE',  ( 6.421262212874594866, -272.7209496839143412, -208.7004858517199750 ) ) ;
#88610=CARTESIAN_POINT ( 'NONE',  ( -96.57482485779813430, -285.1490515983921910, -227.6732145155041280 ) ) ;
#88611=CARTESIAN_POINT ( 'NONE',  ( 30.83068632654069674, -277.3472483584012593, -298.2078099481626623 ) ) ;
#88612=CARTESIAN_POINT ( 'NONE',  ( 24.12559479006556984, -276.9041752298854817, -310.1329236667493205 ) ) ;
#88614=CARTESIAN_POINT ( 'NONE',  ( -104.8891900616303161, -286.9816329611392121, -237.7676025340173283 ) ) ;
#88617=CARTESIAN_POINT ( 'NONE',  ( -58.85335605541897053, -295.1561378050164990, -344.3507737423693129 ) ) ;
#88618=CARTESIAN_POINT ( 'NONE',  ( 16.19194048292264299, -288.7964429797792150, -218.3419280124267914 ) ) ;
#88620=CARTESIAN_POINT ( 'NONE',  ( -19.11405058567864046, -292.3380690714489560, -350.3683826091709648 ) ) ;
#88621=CARTESIAN_POINT ( 'NONE',  ( -96.56989684997603263, -278.1297716425290218, -221.6219857666048085 ) ) ;
#88622=CARTESIAN_POINT ( 'NONE',  ( -95.04166692484002965, -289.6313911323829302, -220.5701624605165989 ) ) ;
#88623=CARTESIAN_POINT ( 'NONE',  ( -111.0029261204034441, -286.1007063871209084, -268.1859085910183467 ) ) ;
#88624=CARTESIAN_POINT ( 'NONE',  ( -109.1498422221659013, -280.0782778267928848, -288.3455259190778861 ) ) ;
#88625=CARTESIAN_POINT ( 'NONE',  ( -2.507841784823749531, -287.9289932179920584, -202.3375934870531694 ) ) ;
#88626=CARTESIAN_POINT ( 'NONE',  ( -18.20129406809804351, -284.8057763877874322, -342.9314820245442661 ) ) ;
#88627=CARTESIAN_POINT ( 'NONE',  ( -3.992928659201691044, -276.7911157575695711, -339.7792152245206125 ) ) ;
#88628=CARTESIAN_POINT ( 'NONE',  ( -76.04232596691096546, -295.5529464540472873, -206.4724589168351656 ) ) ;
#88629=CARTESIAN_POINT ( 'NONE',  ( -97.69557331558651470, -279.0253341055908436, -222.5446982524696296 ) ) ;
#88630=CARTESIAN_POINT ( 'NONE',  ( -111.5322523117048519, -298.3857429496532063, -277.0529540730821623 ) ) ;
#88632=CARTESIAN_POINT ( 'NONE',  ( -4.829096099716510437, -276.9805209788416391, -202.7746430608542312 ) ) ;
#88633=CARTESIAN_POINT ( 'NONE',  ( -36.18366026708313399, -296.2060932151273960, -194.5966729150893286 ) ) ;
#88635=CARTESIAN_POINT ( 'NONE',  ( -109.1049129487920766, -277.8781946815134916, -284.1396437672756861 ) ) ;
#88636=CARTESIAN_POINT ( 'NONE',  ( -4.012810972172158763, -275.6870059649224345, -201.3742721965190299 ) ) ;
#88637=CARTESIAN_POINT ( 'NONE',  ( 19.60089435919962852, -281.3128338431170050, -321.9205309625331211 ) ) ;
#88638=CARTESIAN_POINT ( 'NONE',  ( -64.16755264160346428, -291.1669910849859662, -339.3968251634083799 ) ) ;
#88639=CARTESIAN_POINT ( 'NONE',  ( -100.1907017475590465, -298.6490109233980093, -227.0633194431830191 ) ) ;
#88640=CARTESIAN_POINT ( 'NONE',  ( -35.85324569180153276, -299.2754672156734159, -193.7578905500841415 ) ) ;
#88641=CARTESIAN_POINT ( 'NONE',  ( 35.73471441455897235, -295.3441041765839259, -254.1815934477064047 ) ) ;
#88642=CARTESIAN_POINT ( 'NONE',  ( 35.72509246231228275, -279.7599993724422234, -286.5250361817040243 ) ) ;
#88643=CARTESIAN_POINT ( 'NONE',  ( 1.123503733920095282, -282.4896834319559389, -206.5696595108736631 ) ) ;
#88644=CARTESIAN_POINT ( 'NONE',  ( -82.80461748053576798, -295.5052736394017643, -211.3514467006139057 ) ) ;
#88645=CARTESIAN_POINT ( 'NONE',  ( -112.3458192515958984, -285.9786807552464438, -284.0974308917863596 ) ) ;
#88646=CARTESIAN_POINT ( 'NONE',  ( 18.05009668379463861, -287.1546567275788107, -318.4576719984431179 ) ) ;
#88647=CARTESIAN_POINT ( 'NONE',  ( -69.68305041046212978, -196.9792667690914243, -360.2536513082256420 ) ) ;
#88649=CARTESIAN_POINT ( 'NONE',  ( 12.02124675044623991, -286.9559458369145659, -328.6869764571741257 ) ) ;
#88650=CARTESIAN_POINT ( 'NONE',  ( 25.71216626638022262, -287.7254179250531365, -307.2890142064944712 ) ) ;
#88652=CARTESIAN_POINT ( 'NONE',  ( -65.12732393649616824, -284.4864900801344447, -341.8556918332768646 ) ) ;
#88653=CARTESIAN_POINT ( 'NONE',  ( 32.53785859821213222, -276.1664245850197972, -291.5925520920281997 ) ) ;
#88654=CARTESIAN_POINT ( 'NONE',  ( -22.24114255554162511, -291.1613865355294024, -195.1174766504721561 ) ) ;
#88655=CARTESIAN_POINT ( 'NONE',  ( -4.200242670873950424, -283.2780560982531028, -339.7654770284050301 ) ) ;
#88656=CARTESIAN_POINT ( 'NONE',  ( 24.02254911227997880, -282.4639998806835024, -225.0054494358969919 ) ) ;
#88657=CARTESIAN_POINT ( 'NONE',  ( -34.47550785935203521, -283.3503265921961543, -347.2865964241582333 ) ) ;
#88658=CARTESIAN_POINT ( 'NONE',  ( -87.53062500017432512, -279.3282393588016248, -217.2811494362988753 ) ) ;
#88659=CARTESIAN_POINT ( 'NONE',  ( 10.64812456238590777, -278.1952119285918457, -210.2361428286349110 ) ) ;
#88660=CARTESIAN_POINT ( 'NONE',  ( -109.6919961625490885, -267.3296139387366566, -307.0733402615499017 ) ) ;
#88662=CARTESIAN_POINT ( 'NONE',  ( -3.004098830780497664, -278.5974601216422570, -336.8513997296727780 ) ) ;
#88663=CARTESIAN_POINT ( 'NONE',  ( -13.73103683141038900, -91.22335786429552229, -359.5740944199137061 ) ) ;
#88664=CARTESIAN_POINT ( 'NONE',  ( -34.46657808638739340, -297.4376651245657399, -197.2595125645529492 ) ) ;
#88665=CARTESIAN_POINT ( 'NONE',  ( 17.45018901237726539, -292.3167485788576414, -216.2733541137505426 ) ) ;
#88666=CARTESIAN_POINT ( 'NONE',  ( -29.80965390781157964, -125.3617451572103505, -360.7801904132562640 ) ) ;
#88667=CARTESIAN_POINT ( 'NONE',  ( -3.714752801233152546, -297.0401022983633084, -193.9583019553880092 ) ) ;
#88668=CARTESIAN_POINT ( 'NONE',  ( -70.34836896605899881, -287.8945034334603861, -336.3827083876683446 ) ) ;
#88669=CARTESIAN_POINT ( 'NONE',  ( -15.20223488990918526, -296.6229829561627866, -341.2721600963799347 ) ) ;
#88670=CARTESIAN_POINT ( 'NONE',  ( -72.62538878706820356, -286.8898222516241958, -205.8773942066183338 ) ) ;
#88672=CARTESIAN_POINT ( 'NONE',  ( -95.39567499708275022, -296.8128067305437980, -320.5861736359397014 ) ) ;
#88673=CARTESIAN_POINT ( 'NONE',  ( -73.82208542625367897, -284.0426006330703785, -333.7209790299020824 ) ) ;
#88674=CARTESIAN_POINT ( 'NONE',  ( -9.275710232668592070, -297.1911152518655399, -193.7637831632354164 ) ) ;
#88675=CARTESIAN_POINT ( 'NONE',  ( 21.18080603953344365, -293.6820332346684381, -220.5487007733434552 ) ) ;
#88677=CARTESIAN_POINT ( 'NONE',  ( 22.15767862449141035, -293.3889368381479699, -221.5825280933508736 ) ) ;
#88678=CARTESIAN_POINT ( 'NONE',  ( -89.81779553026244400, -291.4521429466844324, -219.6141041212159166 ) ) ;
#88680=CARTESIAN_POINT ( 'NONE',  ( 18.23474450399076829, -300.6012835206878435, -194.5789127208665263 ) ) ;
#88681=CARTESIAN_POINT ( 'NONE',  ( -18.63202222213688586, -273.0827206845700630, -196.0234190324801489 ) ) ;
#88684=CARTESIAN_POINT ( 'NONE',  ( 24.31458164941571098, -275.6725296414787181, -316.3831759634095420 ) ) ;
#88685=CARTESIAN_POINT ( 'NONE',  ( -109.9126507882185138, -271.1305985069589042, -256.6755721001413235 ) ) ;
#88686=CARTESIAN_POINT ( 'NONE',  ( -108.4164675602245040, -280.6915679219507638, -248.9311642852750595 ) ) ;
#88687=CARTESIAN_POINT ( 'NONE',  ( 21.80698654469597386, -274.3116796373132615, -315.2197665118432610 ) ) ;
#88688=CARTESIAN_POINT ( 'NONE',  ( -107.0889004431211049, -298.0608581902636729, -247.3425335915484595 ) ) ;
#88689=CARTESIAN_POINT ( 'NONE',  ( -35.39605138937105977, -275.0183882440737761, -197.1391267947627455 ) ) ;
#88690=CARTESIAN_POINT ( 'NONE',  ( 7.383749154418845606, -300.2033872413640552, -194.1491647012940405 ) ) ;
#88691=CARTESIAN_POINT ( 'NONE',  ( -90.98020256241385084, -271.3151992230797305, -217.4336406336886398 ) ) ;
#88692=CARTESIAN_POINT ( 'NONE',  ( 24.51793458218403288, -294.7420128473718250, -309.4084772319353647 ) ) ;
#88693=CARTESIAN_POINT ( 'NONE',  ( -70.46985088808011710, -290.1812180999034467, -204.6503841103993580 ) ) ;
#88695=CARTESIAN_POINT ( 'NONE',  ( 24.32209758158868596, -276.6570648336410727, -316.3731050667935847 ) ) ;
#88696=CARTESIAN_POINT ( 'NONE',  ( -43.48424047368110479, -274.1392232603014918, -197.5692963520713192 ) ) ;
#88698=CARTESIAN_POINT ( 'NONE',  ( -99.39836246933839448, -282.6388667859432076, -315.1963967523564065 ) ) ;
#88699=CARTESIAN_POINT ( 'NONE',  ( -60.99002866002962264, -297.3584137180978928, -341.7652595139043115 ) ) ;
#88701=CARTESIAN_POINT ( 'NONE',  ( -72.44252079047399207, -284.7721578009734458, -206.1554842894346677 ) ) ;
#88702=CARTESIAN_POINT ( 'NONE',  ( -27.63470881315206995, -280.9291011480655698, -344.9504649272167285 ) ) ;
#88703=CARTESIAN_POINT ( 'NONE',  ( -37.83875424500602946, -275.2982834352270629, -344.3854110489194795 ) ) ;
#88704=CARTESIAN_POINT ( 'NONE',  ( -3.613444594755383932, -275.1725813218038184, -335.7658555576074946 ) ) ;
#88705=CARTESIAN_POINT ( 'NONE',  ( 37.33900201408090425, -283.4567204032774157, -262.9159391563083545 ) ) ;
#88706=CARTESIAN_POINT ( 'NONE',  ( 33.28410932529845212, -277.0204580825899825, -290.3852732630734295 ) ) ;
#88708=CARTESIAN_POINT ( 'NONE',  ( -110.2655024081480519, -271.2344611497756546, -248.0775304768255296 ) ) ;
#88709=CARTESIAN_POINT ( 'NONE',  ( -66.67116884272201105, -281.6689944626465945, -201.1526597322445298 ) ) ;
#88711=CARTESIAN_POINT ( 'NONE',  ( 24.35490971149054573, -288.8837527053555050, -226.7172366229177953 ) ) ;
#88713=CARTESIAN_POINT ( 'NONE',  ( -57.23126370594855672, -287.3084849448018758, -342.7288532995590344 ) ) ;
#88715=CARTESIAN_POINT ( 'NONE',  ( -102.8800179669123338, -295.7944932136568923, -237.2047042443511202 ) ) ;
#88716=CARTESIAN_POINT ( 'NONE',  ( -110.8493334174409313, -288.5560522963962171, -280.8204182715599018 ) ) ;
#88717=CARTESIAN_POINT ( 'NONE',  ( 192.3098639061998369, 281.3337059592261085, -109.1536320133224081 ) ) ;
#88718=CARTESIAN_POINT ( 'NONE',  ( -55.76085204751009883, -295.8150078359686290, -197.6043155704055323 ) ) ;
#88719=CARTESIAN_POINT ( 'NONE',  ( 34.21087566743413788, -285.6937967938679321, -243.8481655141461033 ) ) ;
#88720=CARTESIAN_POINT ( 'NONE',  ( 1.539924987887209884, -284.1235777564119758, -333.1476651281887484 ) ) ;
#88721=CARTESIAN_POINT ( 'NONE',  ( -98.97982171020632336, -282.1939714606062353, -314.8868599312997389 ) ) ;
#88722=CARTESIAN_POINT ( 'NONE',  ( -72.62694873940402829, -291.5714589620088191, -206.3985147042467361 ) ) ;
#88723=CARTESIAN_POINT ( 'NONE',  ( 31.91525809091074706, -283.3078502666593295, -295.3885569268322797 ) ) ;
#88724=CARTESIAN_POINT ( 'NONE',  ( -34.83078023047895755, -283.8226762067649815, -343.4919586218937297 ) ) ;
#88725=CARTESIAN_POINT ( 'NONE',  ( -7.546561547507297796, -290.6434032765839675, -339.5896251119744989 ) ) ;
#88726=CARTESIAN_POINT ( 'NONE',  ( -3.412640926239523864, -298.6326408371829757, -193.3601811988871759 ) ) ;
#88727=CARTESIAN_POINT ( 'NONE',  ( -56.94140100180641895, -287.3827073712763536, -343.3889323613226452 ) ) ;
#88728=CARTESIAN_POINT ( 'NONE',  ( 25.32690061152271710, -274.9592647916398391, -225.5987980341190848 ) ) ;
#88729=CARTESIAN_POINT ( 'NONE',  ( 9.870087361923538083, -294.6855003705708782, -212.4763284423190726 ) ) ;
#88731=CARTESIAN_POINT ( 'NONE',  ( 21.31550574532285580, -278.6948066931273615, -317.0979686699210447 ) ) ;
#88733=CARTESIAN_POINT ( 'NONE',  ( -100.5690000889176190, -276.0045833875395260, -311.1050903652580359 ) ) ;
#88736=CARTESIAN_POINT ( 'NONE',  ( -37.23404748048368162, -296.4533593876205941, -194.1603856226311393 ) ) ;
#88737=CARTESIAN_POINT ( 'NONE',  ( -63.09882464049199058, -293.3111419126308874, -201.2018022552746288 ) ) ;
#88738=CARTESIAN_POINT ( 'NONE',  ( -100.8021405173969072, -272.3984619785289283, -233.9734640488737796 ) ) ;
#88739=CARTESIAN_POINT ( 'NONE',  ( -110.4752277977036385, -291.9538077196464201, -279.4272573322683684 ) ) ;
#88740=CARTESIAN_POINT ( 'NONE',  ( -41.61852452990174100, -292.9383613026943181, -197.2008026460582641 ) ) ;
#88741=CARTESIAN_POINT ( 'NONE',  ( -109.9270887052928032, -286.5005448722459960, -255.8926909489524633 ) ) ;
#88742=CARTESIAN_POINT ( 'NONE',  ( -8.748681435394530581, -293.8443066618533521, -199.5017814399394354 ) ) ;
#88743=CARTESIAN_POINT ( 'NONE',  ( -71.96417182753269515, -292.9192771186878304, -202.1221085807098348 ) ) ;
#88744=CARTESIAN_POINT ( 'NONE',  ( -4.338558376371498326, -294.4378979190326504, -335.4888061185869219 ) ) ;
#88745=CARTESIAN_POINT ( 'NONE',  ( 11.43478354180057366, -290.3764556504684720, -327.4022150936784783 ) ) ;
#88746=CARTESIAN_POINT ( 'NONE',  ( -0.3735736698964021163, -282.7413115413122568, -337.9212838089801494 ) ) ;
#88747=CARTESIAN_POINT ( 'NONE',  ( -82.09758680927073726, -295.5274530081582043, -209.4173530677898043 ) ) ;
#88748=CARTESIAN_POINT ( 'NONE',  ( -54.96254782434196073, -285.6649382813969851, -195.4044256132371231 ) ) ;
#88749=CARTESIAN_POINT ( 'NONE',  ( 21.97353265476693807, -276.9085197259813071, -225.0239758228853475 ) ) ;
#88750=CARTESIAN_POINT ( 'NONE',  ( -98.42908645621132280, -283.9088561867778253, -229.6737521732676157 ) ) ;
#88751=CARTESIAN_POINT ( 'NONE',  ( 8.972371408197739484, -286.4169884481055419, -329.4187574834333532 ) ) ;
#88752=CARTESIAN_POINT ( 'NONE',  ( -94.02173817196339201, -277.3840602148842436, -220.0850921930528443 ) ) ;
#88754=CARTESIAN_POINT ( 'NONE',  ( -18.72600364087714908, -282.3136698140316980, -341.0637190268167842 ) ) ;
#88755=CARTESIAN_POINT ( 'NONE',  ( -88.67677829477563023, -280.5554650065419082, -213.5041178221238454 ) ) ;
#88756=CARTESIAN_POINT ( 'NONE',  ( 26.16945513870148332, -286.0404186542038474, -227.2197303735168532 ) ) ;
#88757=CARTESIAN_POINT ( 'NONE',  ( 33.72942454330158313, -295.5823839753542188, -291.0675335834604311 ) ) ;
#88758=CARTESIAN_POINT ( 'NONE',  ( -8.171833738087050492, -278.2765967397771192, -340.7709896753364092 ) ) ;
#88759=CARTESIAN_POINT ( 'NONE',  ( -72.59843053132563284, -278.8241603653879679, -338.2746307413582372 ) ) ;
#88760=CARTESIAN_POINT ( 'NONE',  ( -74.01511229425355509, -277.3874166576804896, -333.4805353166745476 ) ) ;
#88761=CARTESIAN_POINT ( 'NONE',  ( -96.75990922141069461, -299.1768040539963067, -224.8484192260559098 ) ) ;
#88762=CARTESIAN_POINT ( 'NONE',  ( 35.50061173354132649, -285.3306234450449210, -253.1584722225344706 ) ) ;
#88763=CARTESIAN_POINT ( 'NONE',  ( -77.69528309073278649, -291.1840553925446784, -335.0603328796804590 ) ) ;
#88764=CARTESIAN_POINT ( 'NONE',  ( 8.410403692695748390, -293.3294014244271466, -327.7061099492979110 ) ) ;
#88765=ORIENTED_EDGE ( 'NONE', *, *, #86805, .F. ) ;
#88766=CARTESIAN_POINT ( 'NONE',  ( 17.09349828530620030, -293.9151031917704131, -319.0512809942784997 ) ) ;
#88768=CARTESIAN_POINT ( 'NONE',  ( -107.4432116647920026, -291.2318458041945632, -301.5926517945230216 ) ) ;
#88769=CARTESIAN_POINT ( 'NONE',  ( -51.85570246182746246, -280.5130522989530277, -198.6627064667482045 ) ) ;
#88770=CARTESIAN_POINT ( 'NONE',  ( -87.87244703221172415, -272.4249887969959900, -212.5023609096001280 ) ) ;
#88771=CARTESIAN_POINT ( 'NONE',  ( 33.76200359271922480, -287.8293561675691308, -240.9376454224967858 ) ) ;
#88772=CARTESIAN_POINT ( 'NONE',  ( -46.01917088447714121, -289.4924822420450141, -346.9024369035943778 ) ) ;
#88773=CARTESIAN_POINT ( 'NONE',  ( -95.78541391206661615, -285.4997418526264710, -226.5841856324762773 ) ) ;
#88774=CARTESIAN_POINT ( 'NONE',  ( 199.3883137936588241, 289.5528945228473958, -97.47147507470964456 ) ) ;
#88775=CARTESIAN_POINT ( 'NONE',  ( 101.5141839819154939, 116.5281249055354067, -281.5031478140604122 ) ) ;
#88776=CARTESIAN_POINT ( 'NONE',  ( -22.13763408965488111, -108.7303330413373033, -358.8740908389603987 ) ) ;
#88777=CARTESIAN_POINT ( 'NONE',  ( -3.802529560586211499, -275.7949203730356658, -335.3820820254225623 ) ) ;
#88778=CARTESIAN_POINT ( 'NONE',  ( -106.7328798081358059, -277.7872383363808240, -246.5602281572855645 ) ) ;
#88779=CARTESIAN_POINT ( 'NONE',  ( -109.1453431151094549, -272.5721129784340064, -242.4658784311463080 ) ) ;
#88780=CARTESIAN_POINT ( 'NONE',  ( -68.85798215598981642, -196.8429261930088217, -357.5647156207587045 ) ) ;
#88781=CARTESIAN_POINT ( 'NONE',  ( -104.5504101214728081, -276.7609001001441129, -306.9163853536769011 ) ) ;
#88782=CARTESIAN_POINT ( 'NONE',  ( -95.81380582698589876, -290.4298608113135742, -314.1884012829152084 ) ) ;
#88783=CARTESIAN_POINT ( 'NONE',  ( -43.28748383492704477, -298.7818394282464283, -193.6998833367696307 ) ) ;
#88784=CARTESIAN_POINT ( 'NONE',  ( -104.1450966862234679, -273.7000923003124058, -232.1672439187108807 ) ) ;
#88785=CARTESIAN_POINT ( 'NONE',  ( -108.4775168079284953, -296.9350704301849646, -253.9691812503791937 ) ) ;
#88788=CARTESIAN_POINT ( 'NONE',  ( -108.3745125533995406, -280.1389628304403914, -296.2755176332486258 ) ) ;
#88789=CARTESIAN_POINT ( 'NONE',  ( -10.72920906819971876, -282.2219963164582737, -342.6070668509094617 ) ) ;
#88790=CARTESIAN_POINT ( 'NONE',  ( -104.7316011881508757, -280.0178595349979673, -241.5023704723153628 ) ) ;
#88791=CARTESIAN_POINT ( 'NONE',  ( -110.3696597728734616, -280.5790546171008373, -249.3637104083806264 ) ) ;
#88792=CARTESIAN_POINT ( 'NONE',  ( -110.2660113002767304, -271.1753318438110227, -259.3945063485154492 ) ) ;
#88793=DIRECTION ( 'NONE',  ( -0.000000000000000000, 1.000000000000000000, 1.224646799147353207E-16 ) ) ;
#88794=CARTESIAN_POINT ( 'NONE',  ( 23.68136368143023773, -281.1622719052827506, -230.2051932776869876 ) ) ;
#88795=CARTESIAN_POINT ( 'NONE',  ( 14.78116627594697974, -277.1431220494483227, -326.8903026726130747 ) ) ;
#88797=CARTESIAN_POINT ( 'NONE',  ( 26.77908828348659753, -277.0297592129062423, -231.3578373895293225 ) ) ;
#88798=CARTESIAN_POINT ( 'NONE',  ( 10.14556184085752832, -274.9870356540658918, -330.2915646690205449 ) ) ;
#88801=CARTESIAN_POINT ( 'NONE',  ( -32.13561320798089582, -291.3166295403516415, -197.3724573444179100 ) ) ;
#88802=CARTESIAN_POINT ( 'NONE',  ( 38.68605035028986094, -286.7551698687362887, -258.7367498470847522 ) ) ;
#88803=CARTESIAN_POINT ( 'NONE',  ( -34.83435733095612363, -281.2601167594040135, -344.3445815098483536 ) ) ;
#88804=CARTESIAN_POINT ( 'NONE',  ( -3.365341808700972770, -281.1691091737433226, -335.6514324568581173 ) ) ;
#88805=CARTESIAN_POINT ( 'NONE',  ( -92.24966424918525831, -291.8367808080635086, -321.5245189587901677 ) ) ;
#88806=CARTESIAN_POINT ( 'NONE',  ( -2.976694331570231444, -281.7219450825382410, -205.4918192799668759 ) ) ;
#88807=CARTESIAN_POINT ( 'NONE',  ( -90.72710357316371699, -271.2949341972904449, -217.6828554168711207 ) ) ;
#88808=CARTESIAN_POINT ( 'NONE',  ( 27.61229810922933581, -280.4792259117083404, -310.3034920856416079 ) ) ;
#88809=CARTESIAN_POINT ( 'NONE',  ( 22.45035533668827199, -296.1715466596770625, -315.6370581208966541 ) ) ;
#88810=CARTESIAN_POINT ( 'NONE',  ( -96.88864188962460844, -277.4321309260640191, -223.1579851984146501 ) ) ;
#88811=CARTESIAN_POINT ( 'NONE',  ( -76.40328641052035152, -278.2407319730143627, -332.2113035366778604 ) ) ;
#88812=CARTESIAN_POINT ( 'NONE',  ( -112.5075799967929555, -286.5567343998617389, -270.0162600337060326 ) ) ;
#88815=CARTESIAN_POINT ( 'NONE',  ( -7.776612193814562701, -294.3566996850324813, -200.8113218426642561 ) ) ;
#88816=CARTESIAN_POINT ( 'NONE',  ( 34.42289870611392644, -273.8333595626176020, -292.1964794839659021 ) ) ;
#88817=CARTESIAN_POINT ( 'NONE',  ( -1.884345576160738389, -287.7917070601843079, -338.5295478394768907 ) ) ;
#88818=CARTESIAN_POINT ( 'NONE',  ( -4.458513102168510933, -290.8927144961657518, -204.2778600655711898 ) ) ;
#88820=CARTESIAN_POINT ( 'NONE',  ( -110.3961455498839968, -277.1260015906198078, -278.8301244749800958 ) ) ;
#88821=CARTESIAN_POINT ( 'NONE',  ( -103.8857275989354463, -294.2517549774662484, -303.3826423662424645 ) ) ;
#88822=CARTESIAN_POINT ( 'NONE',  ( -96.94884573334296363, -291.2701075784368641, -313.3521830034268305 ) ) ;
#88824=CARTESIAN_POINT ( 'NONE',  ( 36.41743059376401703, -291.7844510921906362, -250.7582041716827064 ) ) ;
#88825=CARTESIAN_POINT ( 'NONE',  ( 32.59225633426358115, -288.8425195977143289, -246.7882066578738431 ) ) ;
#88826=CARTESIAN_POINT ( 'NONE',  ( -81.32535161787092193, -289.7029579151109715, -208.3981256949737713 ) ) ;
#88827=CARTESIAN_POINT ( 'NONE',  ( -42.73528288598976133, -287.4080790934755214, -196.9570818155519021 ) ) ;
#88829=CARTESIAN_POINT ( 'NONE',  ( 34.92032093507009449, -288.5065782651537347, -281.8778965209361900 ) ) ;
#88830=CARTESIAN_POINT ( 'NONE',  ( 0.9556996232091388155, -296.5236380136504408, -335.2588527279069694 ) ) ;
#88832=CARTESIAN_POINT ( 'NONE',  ( 37.32910831592712952, -288.5416432545086423, -253.2067829069811182 ) ) ;
#88833=CARTESIAN_POINT ( 'NONE',  ( -100.4986056809782298, -277.1250017337118834, -229.1618528082989030 ) ) ;
#88834=CARTESIAN_POINT ( 'NONE',  ( -35.70770212432291402, -277.3654913112496274, -347.3357499808114994 ) ) ;
#88835=CARTESIAN_POINT ( 'NONE',  ( 26.26554225215162930, -280.6458210426333721, -226.9107153838555178 ) ) ;
#88836=CARTESIAN_POINT ( 'NONE',  ( -87.21761982640481392, -299.3328348492395321, -214.8251887621781577 ) ) ;
#88837=CARTESIAN_POINT ( 'NONE',  ( -87.03269670789117640, -283.3605800741293592, -214.1151700481287321 ) ) ;
#88839=CARTESIAN_POINT ( 'NONE',  ( -54.76000988218859078, -277.9656118216776122, -198.1452542113970594 ) ) ;
#88841=CARTESIAN_POINT ( 'NONE',  ( -27.65628795172891330, -280.9291011470268131, -344.7850856453721917 ) ) ;
#88843=CARTESIAN_POINT ( 'NONE',  ( -56.76639348319081080, -275.7779308852479971, -344.2085583223964704 ) ) ;
#88844=CARTESIAN_POINT ( 'NONE',  ( -76.00549486343447825, -297.0985246431054634, -333.1567060886927152 ) ) ;
#88845=CARTESIAN_POINT ( 'NONE',  ( 21.36448908002214253, -281.1396278516211851, -319.7076057951762778 ) ) ;
#88846=CARTESIAN_POINT ( 'NONE',  ( -108.8189047686954609, -297.2836689099028149, -286.3115933893948295 ) ) ;
#88847=CARTESIAN_POINT ( 'NONE',  ( -46.82599045170345420, -275.3592330692728183, -194.5412358340066135 ) ) ;
#88848=CARTESIAN_POINT ( 'NONE',  ( 11.56383214535435933, -274.4195517779341458, -216.0681613957420950 ) ) ;
#88849=CARTESIAN_POINT ( 'NONE',  ( 31.33128783158213437, -295.9470949734134138, -300.5110992514311192 ) ) ;
#88850=CARTESIAN_POINT ( 'NONE',  ( 31.42084141081734927, -287.2729416256747754, -235.7098137416566601 ) ) ;
#88851=CARTESIAN_POINT ( 'NONE',  ( -100.6707060825276869, -277.1847302277274707, -229.0505764741986638 ) ) ;
#88852=CARTESIAN_POINT ( 'NONE',  ( -111.2315664910461948, -290.6571907444517251, -248.6980698734735142 ) ) ;
#88853=CARTESIAN_POINT ( 'NONE',  ( -101.8560815859694912, -289.1385020599338986, -305.1284889189296337 ) ) ;
#88854=CARTESIAN_POINT ( 'NONE',  ( 35.51102487947743924, -291.7814474102494273, -288.2327787385098645 ) ) ;
#88857=CARTESIAN_POINT ( 'NONE',  ( -110.3067169247177617, -290.1209022522170926, -265.7254710942496558 ) ) ;
#88859=CARTESIAN_POINT ( 'NONE',  ( -93.75499265852629094, -286.2050562525767532, -218.2220763943071233 ) ) ;
#88860=CARTESIAN_POINT ( 'NONE',  ( 22.93080827219366569, -291.9729086501291135, -222.8001783812340761 ) ) ;
#88861=CARTESIAN_POINT ( 'NONE',  ( 37.07265087823328287, -283.0916572806831937, -288.1878883651515366 ) ) ;
#88862=CARTESIAN_POINT ( 'NONE',  ( -2.430530605334753957, -282.4099737776977008, -334.4863285145546570 ) ) ;
#88863=CARTESIAN_POINT ( 'NONE',  ( -98.23397174162738565, -297.1815556975413415, -223.2109593512317645 ) ) ;
#88864=CARTESIAN_POINT ( 'NONE',  ( 13.82809076201679410, -276.1034196780390744, -217.6079571519227329 ) ) ;
#88865=CARTESIAN_POINT ( 'NONE',  ( 9.909078090675439654, -290.7263531353383996, -212.5081523982934186 ) ) ;
#88866=CARTESIAN_POINT ( 'NONE',  ( 9.751543461422579995, -273.5119272719235823, -213.9975088387745075 ) ) ;
#88868=DIRECTION ( 'NONE',  ( -1.000000000000000000, -0.000000000000000000, -0.000000000000000000 ) ) ;
#88869=CARTESIAN_POINT ( 'NONE',  ( 18.84738437295753499, -288.7896401982644079, -221.5338614257992447 ) ) ;
#88870=CARTESIAN_POINT ( 'NONE',  ( -113.8137513682103048, -297.7128243467723792, -263.9102007318877554 ) ) ;
#88871=CARTESIAN_POINT ( 'NONE',  ( -97.44446937599246894, -285.7827541865613625, -228.7270930540353220 ) ) ;
#88872=CARTESIAN_POINT ( 'NONE',  ( -71.47702456065704268, -276.5507692157809174, -339.1186618588110946 ) ) ;
#88873=CARTESIAN_POINT ( 'NONE',  ( -25.04592317527918865, -292.8564399407803762, -194.4524448585611083 ) ) ;
#88874=CARTESIAN_POINT ( 'NONE',  ( 32.88831327036422181, -286.0601276719452244, -298.9269845772616918 ) ) ;
#88875=CARTESIAN_POINT ( 'NONE',  ( 37.07721418950464454, -294.1319605999963755, -290.0479024683017428 ) ) ;
#88876=CARTESIAN_POINT ( 'NONE',  ( -3.630268338155516528, -292.8432786772083887, -205.5874593432622248 ) ) ;
#88879=CARTESIAN_POINT ( 'NONE',  ( 179.9264549738192045, 251.0413663519439638, -164.3140871016692302 ) ) ;
#88881=CARTESIAN_POINT ( 'NONE',  ( -113.4617613181934104, -286.1484793220961933, -264.3225573714302641 ) ) ;
#88882=CARTESIAN_POINT ( 'NONE',  ( -119.3990491898856732, -276.0523547857346784, -270.3284710469131937 ) ) ;
#88884=CARTESIAN_POINT ( 'NONE',  ( -64.18128941018478884, -282.3310806301104776, -338.5803419666793275 ) ) ;
#88885=CARTESIAN_POINT ( 'NONE',  ( -99.63515215918701529, -277.6184400750412351, -315.6081964417838890 ) ) ;
#88886=CARTESIAN_POINT ( 'NONE',  ( 30.62744788623446013, -283.1388142597120918, -238.9285078651561207 ) ) ;
#88887=CARTESIAN_POINT ( 'NONE',  ( 195.4986669975991163, 276.4997496711473559, -124.9842105939577550 ) ) ;
#88888=CARTESIAN_POINT ( 'NONE',  ( -27.46637479669298187, -281.5038967305731603, -346.1840128394300109 ) ) ;
#88889=CARTESIAN_POINT ( 'NONE',  ( 37.08994003297814146, -285.6533146669509620, -276.6443312285128400 ) ) ;
#88890=CARTESIAN_POINT ( 'NONE',  ( -10.80283907500293239, -276.2548437375539265, -199.3405717903672212 ) ) ;
#88891=CARTESIAN_POINT ( 'NONE',  ( -82.39283207028553591, -296.1783962990252235, -327.9441698562145575 ) ) ;
#88892=CARTESIAN_POINT ( 'NONE',  ( 18.86448784015252400, -291.5687922042390596, -223.0102160551004999 ) ) ;
#88893=CARTESIAN_POINT ( 'NONE',  ( -107.4797216441901497, -278.7989106373614732, -302.0179575458226964 ) ) ;
#88894=CARTESIAN_POINT ( 'NONE',  ( -7.507651691420418771, -276.6497464500808405, -336.9864101311050035 ) ) ;
#88895=CARTESIAN_POINT ( 'NONE',  ( -96.70558283186353776, -274.2864917608053474, -221.7873316402643979 ) ) ;
#88896=CARTESIAN_POINT ( 'NONE',  ( -97.69419777710729136, -276.8373959859873139, -317.6799148689655112 ) ) ;
#88897=CARTESIAN_POINT ( 'NONE',  ( -112.7898643569077706, -271.0197764341763218, -296.3298465391314949 ) ) ;
#88898=CARTESIAN_POINT ( 'NONE',  ( 35.34119778660562616, -273.7902327606373092, -288.9104785550536576 ) ) ;
#88899=CARTESIAN_POINT ( 'NONE',  ( 26.03326136535111957, -295.5441535339220422, -313.0485932946843377 ) ) ;
#88901=CARTESIAN_POINT ( 'NONE',  ( 6.757860130087521178, -59.91093500391586701, -350.7441993381422094 ) ) ;
#88902=CARTESIAN_POINT ( 'NONE',  ( -108.6694543714356342, -285.8548569264742696, -253.3784093648953046 ) ) ;
#88903=CARTESIAN_POINT ( 'NONE',  ( -76.21990380771146079, -285.3240072837634784, -335.7096263600781754 ) ) ;
#88904=CARTESIAN_POINT ( 'NONE',  ( -67.58230202556876520, -284.9931624474995715, -203.8073903229725374 ) ) ;
#88905=CARTESIAN_POINT ( 'NONE',  ( -107.1954135973051478, -277.2668652467139054, -246.3946725530375090 ) ) ;
#88906=CARTESIAN_POINT ( 'NONE',  ( -48.49120873738111470, -285.0560121238178226, -343.7542643658638326 ) ) ;
#88907=CARTESIAN_POINT ( 'NONE',  ( -11.48188368726873421, -278.8749462662771066, -201.3000623646655356 ) ) ;
#88908=CARTESIAN_POINT ( 'NONE',  ( 15.83151367117474884, -277.3562006887751750, -320.8272988161273247 ) ) ;
#88910=CARTESIAN_POINT ( 'NONE',  ( -69.52371186195338737, -274.1090396393505557, -204.7691477221953846 ) ) ;
#88911=CARTESIAN_POINT ( 'NONE',  ( 36.44179548098264831, -282.0848744854619667, -248.8627559860956922 ) ) ;
#88912=CARTESIAN_POINT ( 'NONE',  ( 36.92396448756610283, -281.7919726319168490, -250.2079891368959466 ) ) ;
#88916=CARTESIAN_POINT ( 'NONE',  ( 27.62696303721163460, -288.8947537111146744, -231.2807827248599608 ) ) ;
#88917=CARTESIAN_POINT ( 'NONE',  ( -108.3291417091857483, -295.9830231565314875, -252.6071791420796444 ) ) ;
#88918=CARTESIAN_POINT ( 'NONE',  ( -79.53155137547516063, -290.8472859879211114, -206.0064973715321912 ) ) ;
#88919=CARTESIAN_POINT ( 'NONE',  ( 3.987589279887013394, -286.9645246735206001, -331.4357337758737003 ) ) ;
#88920=CARTESIAN_POINT ( 'NONE',  ( -23.69355535698458937, -287.4491842155395602, -342.7257690642406374 ) ) ;
#88921=CARTESIAN_POINT ( 'NONE',  ( -27.95593153036177014, -290.4126423992381660, -196.8938529580860290 ) ) ;
#88922=VECTOR ( 'NONE', #57815, 1000.000000000000000 ) ;
#88923=CARTESIAN_POINT ( 'NONE',  ( 7.155533116394992454, -287.8785201098037305, -211.9263149023260837 ) ) ;
#88924=CARTESIAN_POINT ( 'NONE',  ( -101.8976323444736067, -276.0402284905114243, -308.6406606397787868 ) ) ;
#88925=CARTESIAN_POINT ( 'NONE',  ( -12.50395016080192079, -287.1344564334690972, -342.4547717811892653 ) ) ;
#88926=CARTESIAN_POINT ( 'NONE',  ( 1.678163828981969585, -288.5741197337143262, -206.3107404273475822 ) ) ;
#88927=CARTESIAN_POINT ( 'NONE',  ( -8.949799626988914625, -286.6815371351957538, -339.9733785600924989 ) ) ;
#88928=CARTESIAN_POINT ( 'NONE',  ( 22.78477784429863817, -283.0742888330206597, -312.1727801715958321 ) ) ;
#88929=CARTESIAN_POINT ( 'NONE',  ( -111.9896770885892892, -292.4338905133129742, -279.6047144693898758 ) ) ;
#88930=CARTESIAN_POINT ( 'NONE',  ( 82.14611277039779225, -299.7700546811713593, -193.3686474501289752 ) ) ;
#88932=CARTESIAN_POINT ( 'NONE',  ( -67.62325405607694506, -299.5782460777497249, -201.0786314493083466 ) ) ;
#88933=CARTESIAN_POINT ( 'NONE',  ( -3.064406095733742230, -279.7143613247351368, -205.7120192547222075 ) ) ;
#88934=CARTESIAN_POINT ( 'NONE',  ( 34.66163133151410136, -279.2817490396534481, -249.3725280162958313 ) ) ;
#88935=CARTESIAN_POINT ( 'NONE',  ( 38.19662078253288939, -292.9266175371049030, -284.5077044167479130 ) ) ;
#88936=CARTESIAN_POINT ( 'NONE',  ( -110.8902728777928104, -270.8997547113571613, -262.0797256406096949 ) ) ;
#88937=CARTESIAN_POINT ( 'NONE',  ( -43.34716752544354534, -275.2084350363414273, -344.5584801961832113 ) ) ;
#88938=CARTESIAN_POINT ( 'NONE',  ( -101.8925294664317818, -297.3909674363411568, -305.4956296271776637 ) ) ;
#88940=CARTESIAN_POINT ( 'NONE',  ( -105.0781370570270212, -271.5878690097644039, -234.8860797186684977 ) ) ;
#88941=CARTESIAN_POINT ( 'NONE',  ( -109.3920874496307505, -294.4839957000004347, -294.5006229458841744 ) ) ;
#88942=CARTESIAN_POINT ( 'NONE',  ( 28.00148218434232206, -294.5208031388833092, -236.5137629783081081 ) ) ;
#88945=CARTESIAN_POINT ( 'NONE',  ( 22.71465362648927666, -293.7736288401085289, -228.5558450256074252 ) ) ;
#88947=CARTESIAN_POINT ( 'NONE',  ( -110.1257916780892288, -282.8242249227566845, -250.6490328987756584 ) ) ;
#88948=CARTESIAN_POINT ( 'NONE',  ( -70.93079939629407704, -295.5082394444463034, -335.1884683187761880 ) ) ;
#88949=CARTESIAN_POINT ( 'NONE',  ( -0.3754383079739446183, -282.5746584240786774, -337.9223040882120017 ) ) ;
#88950=CARTESIAN_POINT ( 'NONE',  ( 25.07699156534556195, -282.8988926531994252, -227.6879300705891751 ) ) ;
#88951=CARTESIAN_POINT ( 'NONE',  ( -0.9757982256029431589, -286.1882168460589355, -202.5137490549639665 ) ) ;
#88952=CARTESIAN_POINT ( 'NONE',  ( -104.5017180638011780, -288.1156943239396355, -303.3696080153376897 ) ) ;
#88953=CARTESIAN_POINT ( 'NONE',  ( 37.46200943825348162, -280.2222228821135559, -285.4313797505948287 ) ) ;
#88954=CARTESIAN_POINT ( 'NONE',  ( 7.239277753003735327, -285.3586758794743332, -211.8692464614710218 ) ) ;
#88955=CARTESIAN_POINT ( 'NONE',  ( 34.77707165466368622, -286.8049805708795930, -296.5995496413343631 ) ) ;
#88957=CARTESIAN_POINT ( 'NONE',  ( -55.98594972239119727, -296.8962684004010839, -341.8201798380377454 ) ) ;
#88958=CARTESIAN_POINT ( 'NONE',  ( -98.32213417274323319, -279.3592432990945440, -316.4259674619277121 ) ) ;
#88959=CARTESIAN_POINT ( 'NONE',  ( 14.33207142501330189, -292.3501251635682934, -325.2084345463456998 ) ) ;
#88960=CARTESIAN_POINT ( 'NONE',  ( -14.29818105165613851, -280.0259368854701165, -201.0178091678392320 ) ) ;
#88961=CARTESIAN_POINT ( 'NONE',  ( 38.06147555064014654, -293.5229232442350735, -254.6964678723220743 ) ) ;
#88962=CARTESIAN_POINT ( 'NONE',  ( -98.17016135182011283, -283.2398949312868126, -225.4508232507635910 ) ) ;
#88963=ADVANCED_FACE ( 'NONE', ( #16465 ), #11069, .F. ) ;
#88964=CARTESIAN_POINT ( 'NONE',  ( -23.28802108270996385, -278.8727487968201331, -344.0854311336198066 ) ) ;
#88965=CARTESIAN_POINT ( 'NONE',  ( -55.87439129982982422, -294.3552969704064139, -341.2652627127403662 ) ) ;
#88966=CARTESIAN_POINT ( 'NONE',  ( -112.0379053944801768, -270.6595642647937439, -261.9643719324537869 ) ) ;
#88969=CARTESIAN_POINT ( 'NONE',  ( 29.23731304862225144, -283.0825329258510692, -236.4962975892529187 ) ) ;
#88970=CARTESIAN_POINT ( 'NONE',  ( -90.45628115878515985, -295.3371272909204208, -320.6019992849436449 ) ) ;
#88971=FACE_OUTER_BOUND ( 'NONE', #54804, .T. ) ;
#88972=CARTESIAN_POINT ( 'NONE',  ( -4.771743288812454686, -271.9809262143061233, -202.8022627189028810 ) ) ;
#88973=CARTESIAN_POINT ( 'NONE',  ( 17.98045540647651208, -274.0169670309741150, -216.9591437254168227 ) ) ;
#88974=CARTESIAN_POINT ( 'NONE',  ( 37.80264608039183116, -288.6863896394444282, -255.9866438424649004 ) ) ;
#88975=CARTESIAN_POINT ( 'NONE',  ( -95.76959809118696398, -289.7709401463851009, -314.1447577236851885 ) ) ;
#88976=CARTESIAN_POINT ( 'NONE',  ( -49.27304965492940880, -281.4174497217426278, -197.6400711708310780 ) ) ;
#88977=CARTESIAN_POINT ( 'NONE',  ( -33.77295167291392630, -299.8575643442301839, -196.3466902990889480 ) ) ;
#88978=CARTESIAN_POINT ( 'NONE',  ( -1.760218938713778103, -279.3297746532766155, -206.1654117262181387 ) ) ;
#88980=CARTESIAN_POINT ( 'NONE',  ( -95.08507037260577022, -273.0752038527181185, -219.4228887502702889 ) ) ;
#88981=CARTESIAN_POINT ( 'NONE',  ( -88.94613321542732365, -293.2408207419115342, -216.6400982332671958 ) ) ;
#88983=CARTESIAN_POINT ( 'NONE',  ( -92.63903346802047167, -291.8838965779881391, -222.5479650440476576 ) ) ;
#88985=CARTESIAN_POINT ( 'NONE',  ( 38.47558134905143135, -291.6913957687910397, -270.3344259365086373 ) ) ;
#88987=CARTESIAN_POINT ( 'NONE',  ( -88.13740443269240643, -296.9841929698825425, -217.8321256704426787 ) ) ;
#88989=CARTESIAN_POINT ( 'NONE',  ( -113.4971117055489458, -292.1328764332700416, -265.5589269568019404 ) ) ;
#88990=CARTESIAN_POINT ( 'NONE',  ( -37.30987171927208124, -291.5519495502701375, -350.3611179825600175 ) ) ;
#88991=CARTESIAN_POINT ( 'NONE',  ( 36.80929706736761631, -289.4177090014545115, -259.9010040630292337 ) ) ;
#88992=CARTESIAN_POINT ( 'NONE',  ( 16.90987495324426249, -274.2768656518007901, -321.9052255770073430 ) ) ;
#88993=CARTESIAN_POINT ( 'NONE',  ( -5.943406564085075949, -276.3882997010356917, -202.8669599930505854 ) ) ;
#88994=CARTESIAN_POINT ( 'NONE',  ( 20.47947571497060082, -290.9813570680049111, -223.4578407859972629 ) ) ;
#88995=CARTESIAN_POINT ( 'NONE',  ( -68.19162427447430730, -281.5117552822066500, -201.1473388294926394 ) ) ;
#88997=CARTESIAN_POINT ( 'NONE',  ( -37.54913156659663542, -282.4034372162573732, -343.4752039615685248 ) ) ;
#88998=CARTESIAN_POINT ( 'NONE',  ( -112.4879710563360646, -279.4387047987073061, -285.7403489314895637 ) ) ;
#88999=CARTESIAN_POINT ( 'NONE',  ( -58.39244300135827359, -282.1131718468973304, -344.0700837830037244 ) ) ;
#89000=CARTESIAN_POINT ( 'NONE',  ( -25.79349925096121154, -277.8497269309163471, -346.2522193642396928 ) ) ;
#89002=CARTESIAN_POINT ( 'NONE',  ( 4.466951834050296277, -276.1248781915052177, -206.4647109676793661 ) ) ;
#89003=CARTESIAN_POINT ( 'NONE',  ( -82.13390479932378696, -275.9090924074130271, -214.2458315076590907 ) ) ;
#89005=CARTESIAN_POINT ( 'NONE',  ( -111.3319384704930144, -298.3948235769625512, -282.6267317070384024 ) ) ;
#89006=CARTESIAN_POINT ( 'NONE',  ( -96.80131151909365883, -291.0346430138194478, -313.2421241204754097 ) ) ;
#89007=CARTESIAN_POINT ( 'NONE',  ( -8.117444987741034623, -274.6876243966412972, -339.0611314265431702 ) ) ;
#89008=CARTESIAN_POINT ( 'NONE',  ( -90.86859175108209286, -291.5587617839245809, -324.3688312723742797 ) ) ;
#89009=CARTESIAN_POINT ( 'NONE',  ( 8.919751889117721433, -292.0546183495225705, -213.6935933227010196 ) ) ;
#89010=CARTESIAN_POINT ( 'NONE',  ( 39.57866391366307113, -287.0389200822090174, -268.6924362445642487 ) ) ;
#89012=CARTESIAN_POINT ( 'NONE',  ( -106.9348766131871002, -282.6269174695443667, -295.0741621083533346 ) ) ;
#89013=CARTESIAN_POINT ( 'NONE',  ( -74.13695478333539768, -291.4070181083353077, -334.8503762310150478 ) ) ;
#89014=CARTESIAN_POINT ( 'NONE',  ( -88.15874389209710671, -283.8048174201608731, -216.9913155242664118 ) ) ;
#89015=CARTESIAN_POINT ( 'NONE',  ( -16.79981573297656183, -281.6382884988377100, -199.7971437296610304 ) ) ;
#89016=CARTESIAN_POINT ( 'NONE',  ( -7.001856394474613943, -289.6049309251496311, -340.8899532228931548 ) ) ;
#89017=CARTESIAN_POINT ( 'NONE',  ( -93.99221414101330652, -279.6970203542263107, -224.2231975272558486 ) ) ;
#89018=CARTESIAN_POINT ( 'NONE',  ( -33.54362477606380111, -290.8938937194533878, -193.8524038200291102 ) ) ;
#89019=CARTESIAN_POINT ( 'NONE',  ( 7.441504646455879168, -287.4482362903297599, -207.8566342549276271 ) ) ;
#89020=CARTESIAN_POINT ( 'NONE',  ( -35.15627248501470348, -286.5712146376627629, -193.4405678638204620 ) ) ;
#89021=CARTESIAN_POINT ( 'NONE',  ( -56.31685506482937598, -283.4702369714810288, -340.8518514133517670 ) ) ;
#89024=CARTESIAN_POINT ( 'NONE',  ( -14.26557690012690571, -294.2085436395337865, -198.1409721019649908 ) ) ;
#89025=CARTESIAN_POINT ( 'NONE',  ( 36.97693710062746675, -292.4663230252966173, -288.5828449617946490 ) ) ;
#89026=CARTESIAN_POINT ( 'NONE',  ( -40.52796209958852103, -276.1519098718168834, -343.5395719886201960 ) ) ;
#89027=CARTESIAN_POINT ( 'NONE',  ( -111.5215286208136831, -296.1571202498999469, -249.8995459237500825 ) ) ;
#89028=CARTESIAN_POINT ( 'NONE',  ( 33.29921152532156015, -291.7547796665170949, -249.1953707357953647 ) ) ;
#89029=CARTESIAN_POINT ( 'NONE',  ( -98.02690410923855779, -294.2093275297238506, -312.7318629853191965 ) ) ;
#89030=CARTESIAN_POINT ( 'NONE',  ( -57.78015008514533690, -292.9874789368114989, -199.8139769177015523 ) ) ;
#89031=CARTESIAN_POINT ( 'NONE',  ( 34.63046150111802035, -294.8149008589218170, -284.2979047282708507 ) ) ;
#89033=CARTESIAN_POINT ( 'NONE',  ( -0.3836499478214713266, -292.5618946530282187, -335.8292066949369428 ) ) ;
#89034=CARTESIAN_POINT ( 'NONE',  ( -111.8716590566565827, -298.6656906885456237, -261.5311516812699892 ) ) ;
#89035=CARTESIAN_POINT ( 'NONE',  ( 35.19508572739544405, -288.6272964308869291, -280.5432750523608547 ) ) ;
#89036=CARTESIAN_POINT ( 'NONE',  ( -8.490545543306549092, -278.6562992066666880, -339.9884439290153750 ) ) ;
#89037=CARTESIAN_POINT ( 'NONE',  ( -80.01777561677815243, -276.4102706235498772, -334.0391402479016847 ) ) ;
#89038=CARTESIAN_POINT ( 'NONE',  ( -21.36785844198816520, -273.6004387738561832, -195.1404481632973216 ) ) ;
#89039=CARTESIAN_POINT ( 'NONE',  ( 35.47889646411434228, -279.4314672105670638, -254.8576533790206611 ) ) ;
#89040=CARTESIAN_POINT ( 'NONE',  ( -94.62301593661122467, -276.2648946786512738, -320.6133943071902195 ) ) ;
#89042=CARTESIAN_POINT ( 'NONE',  ( -86.83435579610332411, -294.4429971548641447, -324.6908567253473166 ) ) ;
#89043=CARTESIAN_POINT ( 'NONE',  ( -80.48561767965726688, -275.4679794506541270, -208.9504190740165654 ) ) ;
#89044=CARTESIAN_POINT ( 'NONE',  ( 94.76649097485585571, -300.5504365972934124, -197.1811787442501895 ) ) ;
#89047=CARTESIAN_POINT ( 'NONE',  ( -97.72655729366621813, -287.9592395543290877, -315.4610167626807424 ) ) ;
#89048=CARTESIAN_POINT ( 'NONE',  ( 23.05352618220267757, -274.8149576618262699, -229.3336146960308213 ) ) ;
#89049=CARTESIAN_POINT ( 'NONE',  ( 21.48902162509775948, -288.2214277197815022, -320.0395456750707126 ) ) ;
#89050=CARTESIAN_POINT ( 'NONE',  ( -112.3534138238100581, -274.6237131139723715, -264.7881570981465416 ) ) ;
#89051=CARTESIAN_POINT ( 'NONE',  ( -87.74309054937427277, -293.7581209913942075, -325.6759285460489082 ) ) ;
#89052=CARTESIAN_POINT ( 'NONE',  ( -16.19611019935852525, -281.9828348384396008, -344.2879501172409960 ) ) ;
#89054=CARTESIAN_POINT ( 'NONE',  ( -31.07612613150118008, -280.9729540490905606, -345.1496949390449913 ) ) ;
#89056=CARTESIAN_POINT ( 'NONE',  ( -105.0635442129329249, -289.7262168134909075, -241.9290601960868798 ) ) ;
#89057=CARTESIAN_POINT ( 'NONE',  ( -105.2526652636348388, -282.2949645513912174, -300.3438845652318037 ) ) ;
#89060=CARTESIAN_POINT ( 'NONE',  ( -111.7775110829350496, -288.4340928881269406, -279.5432035619452904 ) ) ;
#89061=CARTESIAN_POINT ( 'NONE',  ( -76.95306132551249334, -275.0310312293645438, -208.2189598626128770 ) ) ;
#89062=CARTESIAN_POINT ( 'NONE',  ( -18.99852665487965453, -284.0263308966909790, -344.7900962463539827 ) ) ;
#89063=CARTESIAN_POINT ( 'NONE',  ( -52.23736057404353517, -271.9428611369167470, -196.2304855949892897 ) ) ;
#89064=CARTESIAN_POINT ( 'NONE',  ( -49.42152875011135649, -285.8939914235181163, -198.3160243476656035 ) ) ;
#89065=CARTESIAN_POINT ( 'NONE',  ( 34.47224366850698374, -277.1884237229274959, -286.4849789586215252 ) ) ;
#89066=CARTESIAN_POINT ( 'NONE',  ( -3.784312916378991254, -277.4003258414024344, -335.3726822687901290 ) ) ;
#89068=CARTESIAN_POINT ( 'NONE',  ( 18.31685722878774669, -284.2537714571871561, -320.7076551815846415 ) ) ;
#89070=CARTESIAN_POINT ( 'NONE',  ( 82.18044315312610593, -297.0737527268180997, -195.3611179825600175 ) ) ;
#89071=CARTESIAN_POINT ( 'NONE',  ( -96.51278045906006753, -295.7225305243627531, -319.6541610964886218 ) ) ;
#89072=CARTESIAN_POINT ( 'NONE',  ( 19.90738172459068522, -288.8668893720492292, -222.4414281454273237 ) ) ;
#89074=CARTESIAN_POINT ( 'NONE',  ( -2.659677404128736544, -292.1237833571632336, -342.4524372437778652 ) ) ;
#89075=CARTESIAN_POINT ( 'NONE',  ( -110.3765361387372508, -277.1751910412162374, -293.9288914978216667 ) ) ;
#89076=CARTESIAN_POINT ( 'NONE',  ( -19.55353988847230085, -290.6769569888583078, -196.2121803957554675 ) ) ;
#89077=CARTESIAN_POINT ( 'NONE',  ( -108.7048720136494637, -286.3126878066204881, -251.9761933834853664 ) ) ;
#89078=CARTESIAN_POINT ( 'NONE',  ( -66.48912589719131461, -281.4252898030412666, -202.3149305971311378 ) ) ;
#89079=CARTESIAN_POINT ( 'NONE',  ( -87.37790602093332382, -286.7958743964533710, -212.5417322798815292 ) ) ;
#89080=CARTESIAN_POINT ( 'NONE',  ( 9.050542965701078302, -284.4160441822205030, -329.3575937758101873 ) ) ;
#89081=CARTESIAN_POINT ( 'NONE',  ( 14.88473760354887077, -276.5070719399959103, -327.0145973572528533 ) ) ;
#89082=CARTESIAN_POINT ( 'NONE',  ( -36.43375537722128854, -296.0836820433624439, -195.7166176068193693 ) ) ;
#89083=CARTESIAN_POINT ( 'NONE',  ( -96.81607964772888408, -279.0426150368054437, -221.4346015617686589 ) ) ;
#89084=CARTESIAN_POINT ( 'NONE',  ( -33.74903269729592381, -300.0176166704152365, -195.9199233160248070 ) ) ;
#89087=CARTESIAN_POINT ( 'NONE',  ( -34.78709695009811753, -296.2233993800615508, -194.5971099260036681 ) ) ;
#89088=DIRECTION ( 'NONE',  ( -1.000000000000000000, -0.000000000000000000, -0.000000000000000000 ) ) ;
#89089=CARTESIAN_POINT ( 'NONE',  ( -59.21939297366914445, -276.8507648694993009, -340.0701919779118612 ) ) ;
#89090=CARTESIAN_POINT ( 'NONE',  ( -78.64046109227615489, -274.7141447982739919, -205.8442902490384085 ) ) ;
#89091=CARTESIAN_POINT ( 'NONE',  ( -3.008861917010193121, -281.6684481228682557, -339.0348577077450045 ) ) ;
#89092=CARTESIAN_POINT ( 'NONE',  ( 18.60604968294815720, -289.9940104596424817, -318.8922244758015268 ) ) ;
#89093=CARTESIAN_POINT ( 'NONE',  ( -110.9583840544445792, -298.3283046013095259, -250.0835621705315646 ) ) ;
#89094=CARTESIAN_POINT ( 'NONE',  ( -94.34577856536363072, -297.0591112527845894, -321.5523650232364616 ) ) ;
#89095=CARTESIAN_POINT ( 'NONE',  ( -14.30564727747010245, -294.3517285953693658, -199.1616187305430969 ) ) ;
#89096=CARTESIAN_POINT ( 'NONE',  ( 35.86385932082201577, -279.3514737473630021, -254.7766081567943672 ) ) ;
#89097=CARTESIAN_POINT ( 'NONE',  ( -39.77227371968641023, -281.9415748106957267, -195.9480388870738068 ) ) ;
#89098=CARTESIAN_POINT ( 'NONE',  ( -80.54429421823286361, -295.5411283990863467, -209.7405764209321148 ) ) ;
#89099=CARTESIAN_POINT ( 'NONE',  ( -104.7341832124922121, -286.6175268055682750, -234.6855518047958640 ) ) ;
#89100=CARTESIAN_POINT ( 'NONE',  ( 25.95603822349596612, -286.9791478944686673, -307.4428225247563660 ) ) ;
#89101=CARTESIAN_POINT ( 'NONE',  ( -111.9029649914729987, -274.3533271841375836, -284.1314302805552643 ) ) ;
#89103=CARTESIAN_POINT ( 'NONE',  ( -7.169427026500634348, -287.2387890439902662, -340.5766734897804326 ) ) ;
#89104=CARTESIAN_POINT ( 'NONE',  ( 15.99281042147283927, -286.5013927213132661, -220.4676463104188997 ) ) ;
#89106=CARTESIAN_POINT ( 'NONE',  ( -13.50490926704745220, -283.8293986118143266, -343.2535038032067973 ) ) ;
#89107=CARTESIAN_POINT ( 'NONE',  ( -16.63873118405083673, -274.6602557992504217, -200.2835814982489637 ) ) ;
#89108=CARTESIAN_POINT ( 'NONE',  ( -39.19040363413979833, -290.9498279827822671, -193.6795311270805939 ) ) ;
#89109=CARTESIAN_POINT ( 'NONE',  ( 39.42797708798034506, -282.2697415680290760, -275.6456175562059343 ) ) ;
#89110=CARTESIAN_POINT ( 'NONE',  ( 31.38848345220755220, -282.6417463983408993, -237.0904182216780214 ) ) ;
#89111=CARTESIAN_POINT ( 'NONE',  ( 29.74555639785409866, -282.3765678172347293, -308.2195247415301083 ) ) ;
#89113=CARTESIAN_POINT ( 'NONE',  ( -39.70123265173319993, -280.0217311979517376, -197.3867410028045697 ) ) ;
#89114=CARTESIAN_POINT ( 'NONE',  ( 17.36665895637873192, -291.6952119285918457, -314.0302885647153062 ) ) ;
#89115=CARTESIAN_POINT ( 'NONE',  ( 204.1738562182569865, 295.5636489450776594, -54.00000000003635847 ) ) ;
#89117=CARTESIAN_POINT ( 'NONE',  ( 37.47532963158331398, -277.5322144758942500, -268.7989139723576955 ) ) ;
#89118=CARTESIAN_POINT ( 'NONE',  ( 193.2878968112678706, 279.2590251747096772, -125.7166890413514722 ) ) ;
#89119=CARTESIAN_POINT ( 'NONE',  ( 26.55706396811117642, -279.0517069514310720, -231.6759935962187740 ) ) ;
#89120=CARTESIAN_POINT ( 'NONE',  ( -108.2718346551197897, -296.1344180275618214, -252.6234966121301966 ) ) ;
#89121=CARTESIAN_POINT ( 'NONE',  ( 8.819018865565656284, -292.1735131886179602, -208.7420833378092482 ) ) ;
#89122=CARTESIAN_POINT ( 'NONE',  ( 122.1069166415481675, 147.2784711292074746, -260.4370888795256178 ) ) ;
#89123=CARTESIAN_POINT ( 'NONE',  ( -29.12011971014949907, -296.7279165062974471, -193.9522893961830619 ) ) ;
#89124=CARTESIAN_POINT ( 'NONE',  ( -66.66544725388411052, -287.8425458187088566, -338.1398679533321570 ) ) ;
#89125=CARTESIAN_POINT ( 'NONE',  ( -101.2174250889782883, -297.9002549988333044, -308.2876331127136496 ) ) ;
#89126=CARTESIAN_POINT ( 'NONE',  ( -77.33135434598976587, -286.8190466279287421, -208.6397927785881734 ) ) ;
#89128=CARTESIAN_POINT ( 'NONE',  ( 26.29112085824403522, -293.9248192799931303, -227.3294859851417300 ) ) ;
#89129=CARTESIAN_POINT ( 'NONE',  ( -96.62842956409112105, -285.6413192482182239, -227.6423237980168324 ) ) ;
#89130=CARTESIAN_POINT ( 'NONE',  ( -70.54299056466236095, -296.4189938815864593, -201.3271912938886601 ) ) ;
#89131=CARTESIAN_POINT ( 'NONE',  ( 6.395908296376385138, -293.4327452979607074, -207.1853280833397832 ) ) ;
#89132=CARTESIAN_POINT ( 'NONE',  ( 39.37923181266253891, -293.9721349783073379, -264.5796384800373175 ) ) ;
#89133=CARTESIAN_POINT ( 'NONE',  ( -31.86923610701748188, -289.1479977434713646, -343.2063299429950121 ) ) ;
#89136=CARTESIAN_POINT ( 'NONE',  ( -37.62717321976086282, -299.9090227726960620, -194.5968520648300739 ) ) ;
#89137=CARTESIAN_POINT ( 'NONE',  ( -85.54640313737958479, -272.1970675487955305, -210.8269653872123115 ) ) ;
#89139=CARTESIAN_POINT ( 'NONE',  ( 35.58783707006125496, -280.5159429295842415, -263.1400257029466729 ) ) ;
#89142=CARTESIAN_POINT ( 'NONE',  ( -39.96713745691275221, -276.5919328570835205, -347.2678273719408821 ) ) ;
#89144=CARTESIAN_POINT ( 'NONE',  ( -51.69734273985348949, -272.2654494168249926, -197.9184609823952599 ) ) ;
#89145=CARTESIAN_POINT ( 'NONE',  ( -65.30296695795047413, -281.5431656365564095, -201.5931527769666900 ) ) ;
#89146=CARTESIAN_POINT ( 'NONE',  ( -35.10373894340448686, -275.1633340817014641, -344.5625803161958061 ) ) ;
#89147=CARTESIAN_POINT ( 'NONE',  ( -58.03132532065379934, -298.9838966303013308, -199.9404540175274576 ) ) ;
#89148=CARTESIAN_POINT ( 'NONE',  ( -107.4251961852876036, -273.7759867085004544, -248.9337898722736497 ) ) ;
#89149=CARTESIAN_POINT ( 'NONE',  ( -107.6291489229502787, -297.7724677766868240, -299.9274261750562687 ) ) ;
#89150=CARTESIAN_POINT ( 'NONE',  ( 14.90517502534841654, -272.8044653843860488, -216.0594528355629222 ) ) ;
#89151=CARTESIAN_POINT ( 'NONE',  ( 31.63899721509572061, -294.5268713193605095, -294.7110019337296762 ) ) ;
#89152=CARTESIAN_POINT ( 'NONE',  ( -28.01381287923609520, -290.7474573783241567, -197.3143058046228759 ) ) ;
#89154=CARTESIAN_POINT ( 'NONE',  ( -87.05065085714393547, -278.2149734987142438, -329.1551525006119050 ) ) ;
#89155=CARTESIAN_POINT ( 'NONE',  ( -110.1889313985378891, -272.7906691278161588, -264.9155664882928249 ) ) ;
#89156=CARTESIAN_POINT ( 'NONE',  ( -81.29204363170602221, -282.3203840553159694, -333.0487810411650003 ) ) ;
#89157=CARTESIAN_POINT ( 'NONE',  ( -33.50238207237256916, -297.0041143795465359, -345.4424805667892997 ) ) ;
#89159=CARTESIAN_POINT ( 'NONE',  ( -78.47583977116995868, -282.8189502839505849, -330.8638805842288662 ) ) ;
#89160=CARTESIAN_POINT ( 'NONE',  ( -37.34047897176560582, -281.0519445899233233, -345.5405427088986698 ) ) ;
#89161=CARTESIAN_POINT ( 'NONE',  ( 27.27552746444510134, -274.6049851869653935, -305.6810719347033114 ) ) ;
#89162=CARTESIAN_POINT ( 'NONE',  ( 22.28025937386015798, -282.9292973018240787, -224.8406054699628385 ) ) ;
#89165=CARTESIAN_POINT ( 'NONE',  ( -69.77257422985915980, -272.0321742184402183, -201.3926766148003082 ) ) ;
#89166=CARTESIAN_POINT ( 'NONE',  ( -98.94795921592940147, -279.9690896066185246, -313.4273143414797573 ) ) ;
#89168=CARTESIAN_POINT ( 'NONE',  ( -36.60451131642521716, -287.9814853994026294, -194.7919155840614280 ) ) ;
#89169=CARTESIAN_POINT ( 'NONE',  ( -112.1113976243086512, -288.4685871173598457, -276.8565991352125479 ) ) ;
#89171=CARTESIAN_POINT ( 'NONE',  ( -96.41080045292979150, -295.9546228856151515, -226.7741858827006638 ) ) ;
#89172=CARTESIAN_POINT ( 'NONE',  ( 16.89752369082219374, -286.4093274500694406, -321.1213341725231771 ) ) ;
#89173=CARTESIAN_POINT ( 'NONE',  ( 164.1991770243031681, 231.0496910105122765, -188.4318802409405009 ) ) ;
#89174=CARTESIAN_POINT ( 'NONE',  ( -104.3069074748270424, -294.9995364145539725, -236.4718762833143728 ) ) ;
#89175=CARTESIAN_POINT ( 'NONE',  ( 37.42503783968690811, -286.2245244606437495, -285.6137455731060868 ) ) ;
#89176=CARTESIAN_POINT ( 'NONE',  ( 27.14814136406135958, -282.6669905289319331, -234.4793571876790281 ) ) ;
#89177=CARTESIAN_POINT ( 'NONE',  ( -85.47797780271102397, -281.9472403570058532, -329.1562945102817821 ) ) ;
#89178=CARTESIAN_POINT ( 'NONE',  ( -110.3062927386186090, -290.5053502780018562, -273.9089570091852011 ) ) ;
#89179=CARTESIAN_POINT ( 'NONE',  ( 36.27639718255356627, -282.9537464046198352, -268.5511185908077323 ) ) ;
#89180=CARTESIAN_POINT ( 'NONE',  ( 27.00190924546948423, -282.8290374801839562, -305.1821125013399865 ) ) ;
#89181=CARTESIAN_POINT ( 'NONE',  ( -81.86019147425703579, -291.6352680838302831, -331.1600548831598871 ) ) ;
#89183=CARTESIAN_POINT ( 'NONE',  ( -51.80269555526009384, -298.0388498572103799, -194.6768926596968754 ) ) ;
#89184=CARTESIAN_POINT ( 'NONE',  ( -23.59831476659382332, -286.9578083656605259, -344.7138382283853275 ) ) ;
#89185=CARTESIAN_POINT ( 'NONE',  ( 37.94539020592240064, -275.3493823729453425, -254.1478096292735813 ) ) ;
#89186=CARTESIAN_POINT ( 'NONE',  ( 17.93970792771565215, -294.8284324881998373, -220.1274613679968297 ) ) ;
#89188=CARTESIAN_POINT ( 'NONE',  ( -4.771743288812468897, -285.1233781216987495, -337.9199732462171255 ) ) ;
#89189=CARTESIAN_POINT ( 'NONE',  ( 27.50124386707673096, -274.0589582039850711, -308.3798112600483137 ) ) ;
#89191=CARTESIAN_POINT ( 'NONE',  ( -112.5962212367760884, -295.1042994807838227, -258.3120809002741112 ) ) ;
#89192=CARTESIAN_POINT ( 'NONE',  ( -95.76001158828768212, -292.7802930512403350, -225.2640969777207545 ) ) ;
#89193=CARTESIAN_POINT ( 'NONE',  ( 17.36735049440609302, -274.2082127979599591, -221.8009234343717537 ) ) ;
#89194=CARTESIAN_POINT ( 'NONE',  ( -109.6149368061015394, -291.8832950641826756, -284.8230446680153705 ) ) ;
#89195=CARTESIAN_POINT ( 'NONE',  ( -60.34420535741542579, -292.6878378045312843, -200.7788218554516675 ) ) ;
#89196=CARTESIAN_POINT ( 'NONE',  ( -96.59041443171668107, -286.9263711691420440, -226.0038878054861300 ) ) ;
#89198=CARTESIAN_POINT ( 'NONE',  ( -58.79080470984933271, -293.2052653879501349, -197.0225728364294184 ) ) ;
#89199=CARTESIAN_POINT ( 'NONE',  ( -16.77538196780092150, -293.6275899025542913, -196.6703802411635706 ) ) ;
#89200=CARTESIAN_POINT ( 'NONE',  ( -6.766841554349227295, -294.4725500585760756, -336.6497144960601418 ) ) ;
#89201=CARTESIAN_POINT ( 'NONE',  ( 20.17971498485812631, -288.8871543923269769, -222.2132946541026683 ) ) ;
#89202=CARTESIAN_POINT ( 'NONE',  ( 39.71043018815907999, -281.7134170121874490, -269.9281493017942921 ) ) ;
#89203=CARTESIAN_POINT ( 'NONE',  ( -113.1056199888904246, -270.7278972505659453, -267.5160169140336848 ) ) ;
#89204=CARTESIAN_POINT ( 'NONE',  ( -113.8193925979152823, -284.4974467066709281, -261.4077633604953235 ) ) ;
#89205=CARTESIAN_POINT ( 'NONE',  ( -6.812378358426629532, -278.6293184499240851, -338.4772490969438650 ) ) ;
#89207=CARTESIAN_POINT ( 'NONE',  ( -100.7518526126499268, -282.8425306519972082, -307.3243844230472064 ) ) ;
#89208=CARTESIAN_POINT ( 'NONE',  ( 12.92580990593084955, -284.7533051498782015, -214.6301393697086439 ) ) ;
#89209=CARTESIAN_POINT ( 'NONE',  ( -97.83179356605262456, -276.0740864099831242, -316.0031827095970129 ) ) ;
#89210=CARTESIAN_POINT ( 'NONE',  ( 144.2857639756989272, -299.5541904835127980, -195.3611179825600175 ) ) ;
#89211=CARTESIAN_POINT ( 'NONE',  ( -94.33695462814144150, -283.4141784266712421, -316.0923928214343164 ) ) ;
#89212=CARTESIAN_POINT ( 'NONE',  ( -112.6089210739956172, -279.9371536216752929, -256.0482047769293104 ) ) ;
#89213=CARTESIAN_POINT ( 'NONE',  ( 14.09812876186115460, -285.8120431873110192, -213.3094072744691232 ) ) ;
#89214=CARTESIAN_POINT ( 'NONE',  ( -7.560276213182880234, -296.4164503735974563, -338.1321056981893207 ) ) ;
#89215=CARTESIAN_POINT ( 'NONE',  ( -98.15255043508705057, -279.5340711093290906, -316.3007241443307862 ) ) ;
#89216=CARTESIAN_POINT ( 'NONE',  ( -4.055898082227022527, -275.7970864155691970, -201.4601768748777602 ) ) ;
#89217=CARTESIAN_POINT ( 'NONE',  ( -97.65002509215020154, -277.8132089877212252, -311.4939022858058593 ) ) ;
#89218=CARTESIAN_POINT ( 'NONE',  ( -104.6999236257464929, -274.9574716888434978, -238.1941080688048089 ) ) ;
#89219=CARTESIAN_POINT ( 'NONE',  ( 36.07802732820382374, -285.7391356277951786, -284.9038503817458263 ) ) ;
#89220=CARTESIAN_POINT ( 'NONE',  ( -54.30350269748556258, -290.8664875480821479, -344.7034651329357757 ) ) ;
#89221=CARTESIAN_POINT ( 'NONE',  ( 19.92665673810715887, -293.1164649939644846, -316.1475025698185277 ) ) ;
#89223=CARTESIAN_POINT ( 'NONE',  ( -57.65675450785669653, -291.4493696423519964, -200.1698916260998544 ) ) ;
#89225=CARTESIAN_POINT ( 'NONE',  ( -9.662020185674874639, -289.7785226143348041, -341.8826380169214190 ) ) ;
#89226=CARTESIAN_POINT ( 'NONE',  ( -104.5390227901078077, -279.5896702800640128, -241.5789621403748981 ) ) ;
#89227=CARTESIAN_POINT ( 'NONE',  ( -113.0820860847279334, -295.6246724429631740, -258.2411397662218064 ) ) ;
#89228=CARTESIAN_POINT ( 'NONE',  ( 30.03823944251314515, -287.7217438255673301, -233.1931772616851788 ) ) ;
#89229=CARTESIAN_POINT ( 'NONE',  ( 20.26810290458961461, -287.1928976206273774, -219.2250679843489820 ) ) ;
#89230=CARTESIAN_POINT ( 'NONE',  ( -110.1164926366131880, -284.8063995113890883, -276.3542025018491586 ) ) ;
#89231=CARTESIAN_POINT ( 'NONE',  ( 153.5330400557857899, 207.2306735197480521, -217.2871232403230408 ) ) ;
#89232=CARTESIAN_POINT ( 'NONE',  ( -114.2273710279701078, -271.6425061313379388, -283.9426671196157486 ) ) ;
#89233=CARTESIAN_POINT ( 'NONE',  ( 160.2329485493519883, 218.0567712857002505, -202.3360275596398310 ) ) ;
#89234=CARTESIAN_POINT ( 'NONE',  ( -70.53517925836121094, -276.6987027068850011, -335.5592365956222807 ) ) ;
#89235=CARTESIAN_POINT ( 'NONE',  ( -78.81816936395172490, -276.5457176553536556, -330.8706733254643382 ) ) ;
#89236=CARTESIAN_POINT ( 'NONE',  ( -58.11182902165122499, -273.4577624967550946, -196.1818530974302064 ) ) ;
#89237=CARTESIAN_POINT ( 'NONE',  ( -46.06860329632770146, -156.0334151122670789, -362.4947484422432353 ) ) ;
#89238=CARTESIAN_POINT ( 'NONE',  ( -23.04756887807354104, -275.5579478501494464, -345.5746246977481633 ) ) ;
#89240=CARTESIAN_POINT ( 'NONE',  ( -71.19570957382865117, -290.0040374636821525, -335.1200932830141710 ) ) ;
#89241=CARTESIAN_POINT ( 'NONE',  ( -3.509142013160955198, -299.2684613794370989, -193.5181099910766420 ) ) ;
#89242=CARTESIAN_POINT ( 'NONE',  ( 35.05613052537813701, -286.0675696423022600, -257.4325782390631048 ) ) ;
#89243=CARTESIAN_POINT ( 'NONE',  ( -31.92121794078451558, -298.6106578659084789, -193.4222168341995598 ) ) ;
#89244=CARTESIAN_POINT ( 'NONE',  ( -3.141877431436876922, -294.7536983832067676, -334.8543124455514430 ) ) ;
#89246=CARTESIAN_POINT ( 'NONE',  ( -12.31953985451911571, -278.6494661464399201, -341.7126099922298295 ) ) ;
#89248=CARTESIAN_POINT ( 'NONE',  ( 37.80406799353948344, -281.2672373653826980, -286.9337652042881928 ) ) ;
#89249=CARTESIAN_POINT ( 'NONE',  ( -96.33360121650478902, -279.0241393913663046, -313.9043519444060735 ) ) ;
#89250=CARTESIAN_POINT ( 'NONE',  ( -67.28834189182781245, -279.1996351473921436, -340.1978752268828430 ) ) ;
#89252=CARTESIAN_POINT ( 'NONE',  ( -50.03788076293803755, -296.4616822065447650, -197.8753820549776208 ) ) ;
#89254=CARTESIAN_POINT ( 'NONE',  ( -11.74513701306266533, -280.5614762424342530, -201.9423488261171826 ) ) ;
#89255=CARTESIAN_POINT ( 'NONE',  ( -15.83238294099916565, -275.1262065567587456, -196.5393191141591274 ) ) ;
#89256=CARTESIAN_POINT ( 'NONE',  ( -75.43933256193851378, -275.5446726038809970, -205.6979167472532879 ) ) ;
#89257=CARTESIAN_POINT ( 'NONE',  ( 28.57838494012721142, -274.6337537995642037, -309.0024000047148434 ) ) ;
#89259=CARTESIAN_POINT ( 'NONE',  ( -108.2624889632463407, -289.9865443180370335, -252.3423510929827671 ) ) ;
#89260=CARTESIAN_POINT ( 'NONE',  ( -113.0381311379151441, -283.7275029288752535, -284.1948195845827740 ) ) ;
#89261=CARTESIAN_POINT ( 'NONE',  ( 26.01516603460677146, -279.2714225129893180, -232.0010455128486626 ) ) ;
#89262=EDGE_CURVE ( 'NONE', #82501, #33611, #14447, .T. ) ;
#89263=CARTESIAN_POINT ( 'NONE',  ( -1.664645030088065525, -279.1096136531650700, -205.9986859479635939 ) ) ;
#89264=CARTESIAN_POINT ( 'NONE',  ( -105.9147152372098617, -283.0148254242084249, -241.2622719470993218 ) ) ;
#89265=CARTESIAN_POINT ( 'NONE',  ( 8.326975155597839517, -290.4277979600607296, -329.9184816361126877 ) ) ;
#89266=CARTESIAN_POINT ( 'NONE',  ( -41.08670985611363591, -281.2090489958015382, -197.0596486410636601 ) ) ;
#89267=CARTESIAN_POINT ( 'NONE',  ( -78.32198314248179827, -208.3160119463293540, -357.0358029796702226 ) ) ;
#89268=CARTESIAN_POINT ( 'NONE',  ( -85.61149910830741305, -282.1072274449032307, -329.3226895339803946 ) ) ;
#89269=CARTESIAN_POINT ( 'NONE',  ( 5.493186313578874547, -296.4728186258708433, -331.9887953628137893 ) ) ;
#89270=CARTESIAN_POINT ( 'NONE',  ( -113.1979372780986495, -276.8484108683283011, -265.9108037149667894 ) ) ;
#89271=CARTESIAN_POINT ( 'NONE',  ( -92.07860617456877605, -285.8317855451488185, -321.8959928985557326 ) ) ;
#89273=CARTESIAN_POINT ( 'NONE',  ( -14.32873870440845998, -294.2682721463203848, -198.3359395594098373 ) ) ;
#89274=CARTESIAN_POINT ( 'NONE',  ( 34.81526441261742377, -273.8157396195682622, -290.8622293634348352 ) ) ;
#89275=CARTESIAN_POINT ( 'NONE',  ( -15.44965522456295304, -285.5255348815132947, -196.6519379049713336 ) ) ;
#89276=CARTESIAN_POINT ( 'NONE',  ( -77.67552561989909066, -289.9004922040765564, -208.5580198783569870 ) ) ;
#89278=CARTESIAN_POINT ( 'NONE',  ( 27.19182294630997987, -274.7150657474394393, -305.6337505060192825 ) ) ;
#89279=CARTESIAN_POINT ( 'NONE',  ( -26.04238081450513320, -293.0463313764469149, -343.7313494206164819 ) ) ;
#89280=CARTESIAN_POINT ( 'NONE',  ( -110.1912367172305238, -291.9994528402514220, -260.2779411251291890 ) ) ;
#89282=CARTESIAN_POINT ( 'NONE',  ( 36.78184658245078253, -292.2614082364067940, -288.5377528565972511 ) ) ;
#89283=CARTESIAN_POINT ( 'NONE',  ( 20.12544109847344487, -288.5044723385692578, -224.0380988027518754 ) ) ;
#89284=CARTESIAN_POINT ( 'NONE',  ( -7.340910553020178142, -286.9039742318146864, -340.1886818209501939 ) ) ;
#89285=CARTESIAN_POINT ( 'NONE',  ( 25.44407166193702352, -288.4527954958793430, -231.9772440623835905 ) ) ;
#89287=CARTESIAN_POINT ( 'NONE',  ( 12.27279899838196719, -289.1433789065411588, -324.1980180626495667 ) ) ;
#89288=CARTESIAN_POINT ( 'NONE',  ( -11.59497176040268585, -296.6985292006157238, -341.2367715873217549 ) ) ;
#89290=CARTESIAN_POINT ( 'NONE',  ( 35.57452106130069325, -289.0540008635130107, -293.8394783572065876 ) ) ;
#89291=CARTESIAN_POINT ( 'NONE',  ( -48.30959273996408854, -275.2703946139339450, -345.1737519845937641 ) ) ;
#89292=CARTESIAN_POINT ( 'NONE',  ( -37.12276323269292533, -277.3827256421054699, -347.3527179268110672 ) ) ;
#89293=CARTESIAN_POINT ( 'NONE',  ( -95.88696434765996912, -278.8934138845136204, -220.3589133636309896 ) ) ;
#89294=CARTESIAN_POINT ( 'NONE',  ( -67.50663542476954149, -299.6344075758300391, -202.0688476716320849 ) ) ;
#89295=CARTESIAN_POINT ( 'NONE',  ( -101.3019709135993196, -283.0784820380062570, -231.0948318536653687 ) ) ;
#89297=CARTESIAN_POINT ( 'NONE',  ( -92.19379891267740845, -277.3971346584839353, -220.3399950438537473 ) ) ;
#89298=CARTESIAN_POINT ( 'NONE',  ( -11.41787826056794941, -280.7144261537449097, -340.7935265535185749 ) ) ;
#89300=CARTESIAN_POINT ( 'NONE',  ( -71.28003470809869668, -275.9719929266736358, -338.7050804172317271 ) ) ;
#89301=CARTESIAN_POINT ( 'NONE',  ( -108.8524076124180624, -298.3056018870816501, -252.5069712928713557 ) ) ;
#89302=CARTESIAN_POINT ( 'NONE',  ( -50.05585669711159369, -282.1309440562471877, -346.0444198705970962 ) ) ;
#89303=CARTESIAN_POINT ( 'NONE',  ( -90.22404417707016933, -298.2228564754190643, -219.6242813242226930 ) ) ;
#89304=CARTESIAN_POINT ( 'NONE',  ( -89.28585022951898509, -298.6546698380873295, -214.1190290492262420 ) ) ;
#89305=CARTESIAN_POINT ( 'NONE',  ( -83.20057052580550305, -273.0704165689758156, -213.5363743181828227 ) ) ;
#89306=CARTESIAN_POINT ( 'NONE',  ( 36.02931961972848285, -295.7527175194100550, -285.9693311777512008 ) ) ;
#89307=CARTESIAN_POINT ( 'NONE',  ( 27.44594658703308099, -288.2658312085144985, -312.0714616590236687 ) ) ;
#89308=CARTESIAN_POINT ( 'NONE',  ( -14.63671863922444416, -278.4238582371012285, -198.2382476489446219 ) ) ;
#89309=CARTESIAN_POINT ( 'NONE',  ( -88.64790453915287571, -291.1886615846689210, -212.9444532116343396 ) ) ;
#89311=CARTESIAN_POINT ( 'NONE',  ( -8.135642908902326553, -287.7188683449310815, -337.5749475652958154 ) ) ;
#89312=CARTESIAN_POINT ( 'NONE',  ( -11.80951754809005827, -290.3842436653737877, -199.7862589130446622 ) ) ;
#89314=CARTESIAN_POINT ( 'NONE',  ( -90.78337343436103879, -230.3218577325732781, -348.1307343985224634 ) ) ;
#89315=CARTESIAN_POINT ( 'NONE',  ( 29.47880164817205895, -287.4586038427289054, -300.0333400375871520 ) ) ;
#89318=CARTESIAN_POINT ( 'NONE',  ( -101.2166761104080450, -284.9301972209697169, -313.0335533777206365 ) ) ;
#89319=CARTESIAN_POINT ( 'NONE',  ( 37.83771883147780812, -292.8056006635608810, -285.8812719355368017 ) ) ;
#89320=CARTESIAN_POINT ( 'NONE',  ( 37.38747727860152992, -283.0744659985058433, -286.8182728805620059 ) ) ;
#89321=CARTESIAN_POINT ( 'NONE',  ( -42.93503437815949297, -282.9578896327762436, -343.1966056410627743 ) ) ;
#89322=CARTESIAN_POINT ( 'NONE',  ( -112.6051595215457297, -296.3487891690641618, -286.6218584370516282 ) ) ;
#89323=CARTESIAN_POINT ( 'NONE',  ( 9.788588059070718828, -276.0317715011957489, -213.9031813598016356 ) ) ;
#89324=CARTESIAN_POINT ( 'NONE',  ( 36.10603311812947425, -291.3995699396595001, -256.9753611624163909 ) ) ;
#89325=CARTESIAN_POINT ( 'NONE',  ( 11.82382920683898675, -273.5478975554822227, -215.7960532026001204 ) ) ;
#89326=ORIENTED_EDGE ( 'NONE', *, *, #48099, .F. ) ;
#89328=CARTESIAN_POINT ( 'NONE',  ( 17.94401428159016021, -288.7721194915838510, -220.4942875993742177 ) ) ;
#89329=CARTESIAN_POINT ( 'NONE',  ( -65.47724550899314977, -296.4911564513986946, -341.7187018202444619 ) ) ;
#89330=CARTESIAN_POINT ( 'NONE',  ( -100.4850125505834768, -284.6987206026236663, -307.1960845805738245 ) ) ;
#89331=CARTESIAN_POINT ( 'NONE',  ( 37.00785565434606639, -274.8507165745961629, -289.4651429160776388 ) ) ;
#89332=CARTESIAN_POINT ( 'NONE',  ( 38.50711987932479019, -294.3631000611373452, -283.1007048759943814 ) ) ;
#89333=CARTESIAN_POINT ( 'NONE',  ( 33.90274207322666911, -286.0243618211891885, -296.2921983274355853 ) ) ;
#89334=CARTESIAN_POINT ( 'NONE',  ( 38.83034196164573615, -293.7419011236542019, -258.8876476171137710 ) ) ;
#89335=CARTESIAN_POINT ( 'NONE',  ( -84.69551565326854359, -290.0589458497315718, -326.0129575035743983 ) ) ;
#89338=CARTESIAN_POINT ( 'NONE',  ( 184.9457000461858911, 260.3766601266518137, -151.0449398723506818 ) ) ;
#89339=CARTESIAN_POINT ( 'NONE',  ( -89.42725907388245332, -286.8548561084268158, -214.5236326855343805 ) ) ;
#89340=CARTESIAN_POINT ( 'NONE',  ( -2.602324593224659921, -277.9809262143061233, -198.2974183793908196 ) ) ;
#89342=CARTESIAN_POINT ( 'NONE',  ( -70.36643853568060081, -282.4183491188379662, -335.8243182341236093 ) ) ;
#89343=CARTESIAN_POINT ( 'NONE',  ( -84.85666301551164281, -277.3535353680069875, -330.9934676387686068 ) ) ;
#89344=CARTESIAN_POINT ( 'NONE',  ( 37.52081958642644111, -283.5285420719779381, -268.5135187135390993 ) ) ;
#89345=CARTESIAN_POINT ( 'NONE',  ( -97.16215191512969795, -248.5819615950344144, -333.1096569481321126 ) ) ;
#89346=CARTESIAN_POINT ( 'NONE',  ( -30.28749668335335343, -281.5392940485725717, -346.4455743865487989 ) ) ;
#89347=CARTESIAN_POINT ( 'NONE',  ( 36.91312325076634693, -285.4739472930680222, -262.7408813532246086 ) ) ;
#89348=CARTESIAN_POINT ( 'NONE',  ( -91.30617101582433293, -275.1548882005277505, -217.1808456871632131 ) ) ;
#89349=CARTESIAN_POINT ( 'NONE',  ( -67.31472652107376575, -295.9484789945013858, -337.0052044219577851 ) ) ;
#89351=CARTESIAN_POINT ( 'NONE',  ( -38.89129835274776781, -290.7171322168924235, -196.8843037843466846 ) ) ;
#89352=CARTESIAN_POINT ( 'NONE',  ( -75.27868253275025268, -278.1955923387690177, -337.2498177208484549 ) ) ;
#89353=CARTESIAN_POINT ( 'NONE',  ( 34.37350040502551707, -275.3722757485521129, -256.7255023933661278 ) ) ;
#89354=CARTESIAN_POINT ( 'NONE',  ( 30.98117113246196297, -274.0220486065021532, -235.5261101369746370 ) ) ;
#89356=CARTESIAN_POINT ( 'NONE',  ( -0.5964661703469381626, -272.5401866390137116, -204.9646677080317545 ) ) ;
#89357=CARTESIAN_POINT ( 'NONE',  ( -50.34922146392676723, -296.6402220358645536, -345.7101376294679085 ) ) ;
#89360=CARTESIAN_POINT ( 'NONE',  ( -109.4997218494661837, -285.8027373141791827, -257.3503336445327818 ) ) ;
#89361=CARTESIAN_POINT ( 'NONE',  ( -98.95351071658519970, -285.7136852403548346, -314.9232657090777820 ) ) ;
#89362=CARTESIAN_POINT ( 'NONE',  ( -102.3252208087818644, -284.3552683475984963, -236.8792615856718555 ) ) ;
#89363=CARTESIAN_POINT ( 'NONE',  ( -48.75141068166987424, -275.5995907636105926, -343.3257522533755264 ) ) ;
#89364=CARTESIAN_POINT ( 'NONE',  ( 22.01152033341270808, -284.0284413453724142, -314.9698065617142220 ) ) ;
#89365=CARTESIAN_POINT ( 'NONE',  ( -109.1663451174775474, -276.8158102312803521, -286.9073476630500750 ) ) ;
#89367=CARTESIAN_POINT ( 'NONE',  ( 13.95741670306516902, -277.3916214387619448, -322.8019233444435372 ) ) ;
#89370=CARTESIAN_POINT ( 'NONE',  ( -45.26690633183829249, -280.7571534642659685, -193.8795140799045100 ) ) ;
#89371=CARTESIAN_POINT ( 'NONE',  ( 8.504836755616295818, -281.1533043670194161, -208.5079879935735789 ) ) ;
#89375=CARTESIAN_POINT ( 'NONE',  ( 38.11935580131428480, -289.4987117615590364, -277.1386187615212862 ) ) ;
#89376=CARTESIAN_POINT ( 'NONE',  ( -109.9660671430326886, -295.6274957326057802, -279.6161511934201940 ) ) ;
#89377=CARTESIAN_POINT ( 'NONE',  ( -111.5322591558799417, -290.1549628184417315, -250.0856013454351796 ) ) ;
#89378=CARTESIAN_POINT ( 'NONE',  ( 5.327607962648773565, -284.8778091894870954, -209.8227397338502556 ) ) ;
#89379=CARTESIAN_POINT ( 'NONE',  ( 28.19106208172495798, -285.6743395057474686, -236.7698823458048594 ) ) ;
#89380=CARTESIAN_POINT ( 'NONE',  ( -108.7088430292875216, -288.5341825606834618, -290.1640951390168652 ) ) ;
#89381=CARTESIAN_POINT ( 'NONE',  ( -62.71446410875797284, -286.9196287641611889, -201.4349049733087043 ) ) ;
#89382=CARTESIAN_POINT ( 'NONE',  ( -109.5228071251508055, -276.2899097199914422, -290.7299285319364799 ) ) ;
#89383=CARTESIAN_POINT ( 'NONE',  ( -48.76935568181369263, -287.5950964036263713, -345.7527351328146779 ) ) ;
#89384=CARTESIAN_POINT ( 'NONE',  ( -32.46264471921647043, -288.1138060280721334, -195.5071587187340185 ) ) ;
#89385=CARTESIAN_POINT ( 'NONE',  ( -31.98351722481240245, -286.9846679679006911, -345.3878743078071807 ) ) ;
#89387=CARTESIAN_POINT ( 'NONE',  ( -24.01094357624661413, -283.8189348993204817, -342.3729182461612481 ) ) ;
#89388=CARTESIAN_POINT ( 'NONE',  ( -103.5293050178018603, -292.0804366665715293, -305.9873636831243289 ) ) ;
#89391=CARTESIAN_POINT ( 'NONE',  ( -102.6183485460080647, -298.9780851594219939, -232.2017639280127526 ) ) ;
#89392=CARTESIAN_POINT ( 'NONE',  ( -1.878874007633794418, -279.7319528412278373, -206.3690115102664038 ) ) ;
#89393=CARTESIAN_POINT ( 'NONE',  ( 27.26939882073375543, -280.0623675382756801, -308.5478871368379714 ) ) ;
#89394=CARTESIAN_POINT ( 'NONE',  ( -19.33506313426462242, -294.0234935300373991, -345.1147478915953002 ) ) ;
#89395=CARTESIAN_POINT ( 'NONE',  ( 52.91742506675634417, -297.6002664758410674, -196.5862250154463027 ) ) ;
#89396=CARTESIAN_POINT ( 'NONE',  ( 32.69620998941175571, -280.5322213171500607, -292.7963291489726316 ) ) ;
#89397=CARTESIAN_POINT ( 'NONE',  ( -0.7839563394423398890, -274.6428808302404718, -335.2642193749258013 ) ) ;
#89398=CARTESIAN_POINT ( 'NONE',  ( -80.43046367778833883, -296.9652166222387564, -329.8976776119802139 ) ) ;
#89400=CARTESIAN_POINT ( 'NONE',  ( -108.6104089258873415, -271.4802977088584157, -242.6587614327106905 ) ) ;
#89401=CARTESIAN_POINT ( 'NONE',  ( -22.32008223769805255, -293.1021836508136857, -344.8481974480610006 ) ) ;
#89402=CARTESIAN_POINT ( 'NONE',  ( -25.33065611174975018, -293.6333903884172400, -197.7068171634307703 ) ) ;
#89404=CARTESIAN_POINT ( 'NONE',  ( 33.80239623952288497, -294.1297444140612924, -253.2454116158244233 ) ) ;
#89406=CARTESIAN_POINT ( 'NONE',  ( -60.74530722553166129, -281.3742846077544755, -342.0443710660948682 ) ) ;
#89407=CARTESIAN_POINT ( 'NONE',  ( -68.51733844332717638, -295.4735227503932151, -336.3830273528693624 ) ) ;
#89408=CARTESIAN_POINT ( 'NONE',  ( 25.93032726673651567, -282.1321097808176432, -314.2665421819561402 ) ) ;
#89409=CARTESIAN_POINT ( 'NONE',  ( 31.84442904996111068, -283.0775418811463737, -239.9868900143509620 ) ) ;
#89410=CARTESIAN_POINT ( 'NONE',  ( -43.66029834974155932, -285.6412345998592173, -193.5887780097785935 ) ) ;
#89411=CARTESIAN_POINT ( 'NONE',  ( -94.83234444130621910, -289.2152406181785409, -222.4364852949967428 ) ) ;
#89412=CARTESIAN_POINT ( 'NONE',  ( -13.65569264099284652, -281.2300240906441786, -342.8985621121468625 ) ) ;
#89413=CARTESIAN_POINT ( 'NONE',  ( 28.10487465666762930, -285.7844200708175322, -236.8125148771269437 ) ) ;
#89414=CARTESIAN_POINT ( 'NONE',  ( 35.64932073798920698, -286.7696222920217224, -293.8941454666069149 ) ) ;
#89416=CARTESIAN_POINT ( 'NONE',  ( -67.60483385280748792, -297.0560810212458591, -337.6845789042358206 ) ) ;
#89417=CARTESIAN_POINT ( 'NONE',  ( 23.06348465569197614, -277.6072768240239270, -317.1778564322460738 ) ) ;
#89418=CARTESIAN_POINT ( 'NONE',  ( -67.58959721577458879, -293.4671412832298643, -339.3790252758977317 ) ) ;
#89419=CARTESIAN_POINT ( 'NONE',  ( -85.49494253552357748, -279.0308847195248632, -215.4671043532024157 ) ) ;
#89420=CARTESIAN_POINT ( 'NONE',  ( 38.85158054002001649, -293.5753268677494816, -258.8865971006352424 ) ) ;
#89421=CARTESIAN_POINT ( 'NONE',  ( -64.01553590476950717, -283.7868149177917871, -199.6519509270303274 ) ) ;
#89422=CARTESIAN_POINT ( 'NONE',  ( -12.50385522402253713, -278.7294596734267884, -341.1834041075422306 ) ) ;
#89423=CARTESIAN_POINT ( 'NONE',  ( -78.09058255606841215, -294.6732798875499384, -331.2741399715538932 ) ) ;
#89424=CARTESIAN_POINT ( 'NONE',  ( -111.7261818921962657, -270.6950922534273900, -259.1913258926078356 ) ) ;
#89427=CARTESIAN_POINT ( 'NONE',  ( 29.63786612094960304, -283.9700359865263977, -303.4267081921054228 ) ) ;
#89428=CARTESIAN_POINT ( 'NONE',  ( 8.261691419512516177, -293.9166311337340289, -327.5078217727971150 ) ) ;
#89429=DIRECTION ( 'NONE',  ( 0.000000000000000000, 0.000000000000000000, -1.000000000000000000 ) ) ;
#89430=CARTESIAN_POINT ( 'NONE',  ( -110.4542110544635705, -270.2666405000204009, -253.6410175316879361 ) ) ;
#89431=CARTESIAN_POINT ( 'NONE',  ( -102.5765401351289086, -272.2816307452516185, -229.7584768185925554 ) ) ;
#89432=CARTESIAN_POINT ( 'NONE',  ( 7.658067293608112891, -289.7677158402987629, -332.2998705699396282 ) ) ;
#89433=CARTESIAN_POINT ( 'NONE',  ( -18.47555092028106571, -288.6357094860068742, -340.9336893357166787 ) ) ;
#89434=CARTESIAN_POINT ( 'NONE',  ( -72.47715935342125704, -281.0982339343012200, -205.5829792430650969 ) ) ;
#89435=CARTESIAN_POINT ( 'NONE',  ( -111.1417001269576588, -274.1520230526816704, -270.3814443024369325 ) ) ;
#89436=CARTESIAN_POINT ( 'NONE',  ( -49.19098065889696159, -278.6926907910788600, -197.9268370460091546 ) ) ;
#89438=CARTESIAN_POINT ( 'NONE',  ( -78.18764879069254903, -297.1854389532834375, -205.1127251338899100 ) ) ;
#89439=CARTESIAN_POINT ( 'NONE',  ( -25.19779744363221141, -294.1281924848746030, -196.8658608858496564 ) ) ;
#89440=CARTESIAN_POINT ( 'NONE',  ( 30.18048445740676300, -294.6905496191523071, -234.9319349767842198 ) ) ;
#89441=PLANE ( 'NONE',  #50658 ) ;
#89442=CARTESIAN_POINT ( 'NONE',  ( -98.38922950490488972, -291.7615813757562364, -230.0560744510994198 ) ) ;
#89444=CARTESIAN_POINT ( 'NONE',  ( -53.10876038268776966, -289.9918161514729604, -196.2014567411923451 ) ) ;
#89446=CARTESIAN_POINT ( 'NONE',  ( -44.56695475053873423, -297.6250690021802825, -197.6479168033173437 ) ) ;
#89447=CARTESIAN_POINT ( 'NONE',  ( 132.9888089158688445, -299.5541904835127980, -202.0104999926936387 ) ) ;
#89450=CARTESIAN_POINT ( 'NONE',  ( -100.0992595278448505, -291.4937834876097895, -313.7684502109029268 ) ) ;
#89451=CARTESIAN_POINT ( 'NONE',  ( -55.63300648810263738, -294.3376638359845288, -190.3683826091709363 ) ) ;
#89452=CARTESIAN_POINT ( 'NONE',  ( -8.817577174657690975, -288.4263100684626124, -201.1634395857448396 ) ) ;
#89453=CARTESIAN_POINT ( 'NONE',  ( -8.234802571833906626, -272.4338772165622231, -201.3651656009776616 ) ) ;
#89454=CARTESIAN_POINT ( 'NONE',  ( 18.34686840596227952, -276.7793647409547475, -220.8874262223460505 ) ) ;
#89455=CARTESIAN_POINT ( 'NONE',  ( -6.654716109768185284, -290.5380812150057181, -202.5405959210113451 ) ) ;
#89456=CARTESIAN_POINT ( 'NONE',  ( -74.42438996437691401, -281.4247891971587592, -204.2916121887988083 ) ) ;
#89458=CARTESIAN_POINT ( 'NONE',  ( 20.25616722230283884, -281.5343718934914250, -315.3764303245428096 ) ) ;
#89459=CARTESIAN_POINT ( 'NONE',  ( -112.1034855576187113, -279.8464499182607028, -253.2681969077653150 ) ) ;
#89460=CARTESIAN_POINT ( 'NONE',  ( -6.376732243084020979, -279.2448364066792692, -200.2813807390731426 ) ) ;
#89461=CARTESIAN_POINT ( 'NONE',  ( -95.25716805911793017, -238.2204399489505136, -338.9131918094142293 ) ) ;
#89462=CARTESIAN_POINT ( 'NONE',  ( 35.50286416067508100, -276.1857100173000390, -245.9760889050689627 ) ) ;
#89464=CARTESIAN_POINT ( 'NONE',  ( 19.50628162436637325, -276.3748997461619865, -219.3814804009799673 ) ) ;
#89465=CARTESIAN_POINT ( 'NONE',  ( -85.33152481854864391, -299.9090924074131408, -210.2361428286349110 ) ) ;
#89468=CARTESIAN_POINT ( 'NONE',  ( -98.36037189802839009, -291.0698786233921851, -311.0158215604650991 ) ) ;
#89469=CARTESIAN_POINT ( 'NONE',  ( -84.51777558273262514, -291.4513693691804406, -329.9966162680774460 ) ) ;
#89470=CARTESIAN_POINT ( 'NONE',  ( 6.744307514924360980, -292.0187043061973213, -212.0488842923588493 ) ) ;
#89471=CARTESIAN_POINT ( 'NONE',  ( 20.24486260099647339, -286.3674025849967393, -219.2597765706826181 ) ) ;
#89473=CARTESIAN_POINT ( 'NONE',  ( -32.10909449115905545, -281.3849132347797877, -343.9753846289269745 ) ) ;
#89474=CARTESIAN_POINT ( 'NONE',  ( 36.18706099546115951, -289.5463120928164926, -280.6708646512282712 ) ) ;
#89475=CARTESIAN_POINT ( 'NONE',  ( 19.01216452693342163, -280.7004775883492584, -317.8670106553200299 ) ) ;
#89477=CARTESIAN_POINT ( 'NONE',  ( -14.16916049563535651, -281.6741265309902360, -200.5629539912193309 ) ) ;
#89478=CARTESIAN_POINT ( 'NONE',  ( 22.23015896804160718, -289.1451100435464809, -318.7968261610265586 ) ) ;
#89479=CARTESIAN_POINT ( 'NONE',  ( -87.57748483340623125, -279.8205072657860910, -217.2407063370519893 ) ) ;
#89480=CARTESIAN_POINT ( 'NONE',  ( 6.282760694807794977, -291.4251603220413926, -207.3935458872689708 ) ) ;
#89481=CARTESIAN_POINT ( 'NONE',  ( 24.56709055569362121, -287.7491371279205623, -224.8478182016912399 ) ) ;
#89482=CARTESIAN_POINT ( 'NONE',  ( 9.768125325348606225, -287.1736571232110578, -209.5319206444170561 ) ) ;
#89483=CARTESIAN_POINT ( 'NONE',  ( -38.88295117023228897, -283.2386657512871579, -343.3573368668735384 ) ) ;
#89486=CARTESIAN_POINT ( 'NONE',  ( -33.62405605891816407, -293.9588901553893834, -194.6875783233080597 ) ) ;
#89487=CARTESIAN_POINT ( 'NONE',  ( 35.82032427846419154, -291.9542323640077370, -247.9866580422593927 ) ) ;
#89488=CARTESIAN_POINT ( 'NONE',  ( 22.65171675344419810, -275.1958268891521016, -312.4505239295602905 ) ) ;
#89489=CARTESIAN_POINT ( 'NONE',  ( -106.4181144413962414, -296.3352296150459892, -236.5711524323585309 ) ) ;
#89490=CARTESIAN_POINT ( 'NONE',  ( 0.2794937784735365693, -291.0429634010310451, -206.9943007867879032 ) ) ;
#89491=CARTESIAN_POINT ( 'NONE',  ( -110.3663237032401696, -294.6351290922206658, -282.4184131245139611 ) ) ;
#89492=CARTESIAN_POINT ( 'NONE',  ( -17.33904456994252996, -293.5210522161517588, -199.6893769056655401 ) ) ;
#89493=CARTESIAN_POINT ( 'NONE',  ( -9.623295292990453831, -293.5025586904683905, -202.4402105184946947 ) ) ;
#89495=CARTESIAN_POINT ( 'NONE',  ( -50.18006202488202661, -293.2153406335911541, -344.4759498966058118 ) ) ;
#89496=CARTESIAN_POINT ( 'NONE',  ( -40.56572100135387160, -300.0117644542553421, -195.4272741709044112 ) ) ;
#89497=CARTESIAN_POINT ( 'NONE',  ( 23.71225731600947739, -289.0530819438629919, -310.8293345781241328 ) ) ;
#89498=CARTESIAN_POINT ( 'NONE',  ( 27.68949517821442186, -278.0383698159658934, -308.4314533864418308 ) ) ;
#89499=CARTESIAN_POINT ( 'NONE',  ( -99.33748818300107075, -276.7467863792031153, -315.3782167805674135 ) ) ;
#89500=CARTESIAN_POINT ( 'NONE',  ( -85.73764015344455913, -272.7506409636969806, -210.6020536045909353 ) ) ;
#89501=CARTESIAN_POINT ( 'NONE',  ( 35.98978329911530949, -279.4664256948481693, -257.5623782858217510 ) ) ;
#89502=CARTESIAN_POINT ( 'NONE',  ( -88.68823285611243534, -276.1585796520872691, -326.6636400448284689 ) ) ;
#89503=CARTESIAN_POINT ( 'NONE',  ( -109.2582484549825921, -295.4361481255918989, -255.1595544451657531 ) ) ;
#89505=CARTESIAN_POINT ( 'NONE',  ( -69.54332678119122590, -274.2680799018471589, -204.7337768093673276 ) ) ;
#89508=CARTESIAN_POINT ( 'NONE',  ( -96.02541180810462151, -287.9245676861992251, -317.6533354294903120 ) ) ;
#89509=CARTESIAN_POINT ( 'NONE',  ( -64.56681560066327563, -273.5199108060260755, -202.6143888029167499 ) ) ;
#89511=CARTESIAN_POINT ( 'NONE',  ( 7.934511617521064153, -288.4527535073499394, -332.7090066298840725 ) ) ;
#89512=CARTESIAN_POINT ( 'NONE',  ( -109.2899178662530915, -274.8341690076491659, -248.4233425930360681 ) ) ;
#89513=CARTESIAN_POINT ( 'NONE',  ( -95.38019244579690792, -293.8995456241070201, -317.6206749504253253 ) ) ;
#89515=CARTESIAN_POINT ( 'NONE',  ( -35.91247187751956460, -282.2318601589695390, -347.1994386176735929 ) ) ;
#89518=CARTESIAN_POINT ( 'NONE',  ( -12.13826047484608139, -280.7241860383239782, -341.0534281199036286 ) ) ;
#89520=CARTESIAN_POINT ( 'NONE',  ( -102.7565311824030942, -289.7980703111861658, -236.9615677730293442 ) ) ;
#89521=CARTESIAN_POINT ( 'NONE',  ( -76.80346382140157857, -281.7257616959386155, -333.2998574769731590 ) ) ;
#89524=CARTESIAN_POINT ( 'NONE',  ( -106.5387474176101250, -288.9312600503197928, -241.2991152413904388 ) ) ;
#89525=CARTESIAN_POINT ( 'NONE',  ( -16.46258788178147370, -275.8469055298156150, -199.6342240971159185 ) ) ;
#89526=CARTESIAN_POINT ( 'NONE',  ( -85.83907311387635275, -284.9119800860808596, -329.6571004007793135 ) ) ;
#89527=CARTESIAN_POINT ( 'NONE',  ( -65.66433593259694135, -271.7645022383798050, -200.2962157397798819 ) ) ;
#89528=CARTESIAN_POINT ( 'NONE',  ( -103.0126648816664812, -284.1191776638242459, -302.3570525356987559 ) ) ;
#89529=CARTESIAN_POINT ( 'NONE',  ( 36.17457843463265732, -276.9214979134900432, -266.0867995092721117 ) ) ;
#89530=CARTESIAN_POINT ( 'NONE',  ( -1.381964546635444435, -277.3654279028797305, -334.1326485075859409 ) ) ;
#89531=CARTESIAN_POINT ( 'NONE',  ( 31.73412386079864334, -283.9355731619110088, -299.7091107255139946 ) ) ;
#89534=CARTESIAN_POINT ( 'NONE',  ( 37.78345704703205143, -293.5974273715423806, -287.3088078472175084 ) ) ;
#89535=CARTESIAN_POINT ( 'NONE',  ( 33.83452654890530908, -289.2399818291281690, -247.8285627679293555 ) ) ;
#89537=CARTESIAN_POINT ( 'NONE',  ( -111.2586520408596868, -294.4809262143061801, -234.7283546768995564 ) ) ;
#89538=CARTESIAN_POINT ( 'NONE',  ( -111.2879077670209540, -277.4870441926948388, -291.2445371603733975 ) ) ;
#89539=CARTESIAN_POINT ( 'NONE',  ( -3.656448422669502207, -290.8890959978990054, -201.9965700247914242 ) ) ;
#89541=CARTESIAN_POINT ( 'NONE',  ( -108.0254573401965388, -286.3475910243426483, -249.3389682291132772 ) ) ;
#89542=CARTESIAN_POINT ( 'NONE',  ( -0.9527373633970337430, -278.3225820091101923, -334.8692371559108096 ) ) ;
#89543=CARTESIAN_POINT ( 'NONE',  ( -3.764777859138308980, -287.9117285792387975, -201.7085463397041281 ) ) ;
#89544=CARTESIAN_POINT ( 'NONE',  ( 36.19661376582089929, -283.7423361385128260, -285.1607479984036218 ) ) ;
#89545=CARTESIAN_POINT ( 'NONE',  ( 36.88618722070909683, -275.9758810718828954, -290.8851671381925712 ) ) ;
#89546=CARTESIAN_POINT ( 'NONE',  ( -41.38656795465438165, -276.9350503042121545, -347.2680134802552629 ) ) ;
#89547=CARTESIAN_POINT ( 'NONE',  ( -37.17037521643547393, -299.9744739958862851, -195.9181485666683216 ) ) ;
#89549=CARTESIAN_POINT ( 'NONE',  ( -35.48537860860557203, -296.2147462987906010, -194.5968914209361458 ) ) ;
#89551=CARTESIAN_POINT ( 'NONE',  ( -104.3303182376368881, -277.6664958076602829, -299.6514788180591040 ) ) ;
#89552=CARTESIAN_POINT ( 'NONE',  ( -91.89709851682771102, -274.4996536539099452, -216.5864285385212611 ) ) ;
#89553=CARTESIAN_POINT ( 'NONE',  ( 38.95033447754254041, -280.4983550037198370, -261.3894040300933739 ) ) ;
#89554=CARTESIAN_POINT ( 'NONE',  ( 30.88732767148243497, -288.9310968579018208, -241.5444558237892352 ) ) ;
#89555=CARTESIAN_POINT ( 'NONE',  ( -90.21755856913489424, -297.3033715790449492, -325.4506740825601128 ) ) ;
#89556=CARTESIAN_POINT ( 'NONE',  ( -58.72568541237021122, -296.5276727506683869, -343.9740910476299973 ) ) ;
#89557=CARTESIAN_POINT ( 'NONE',  ( -22.39883148805939328, -294.2441040339019764, -197.0348668834258206 ) ) ;
#89558=CARTESIAN_POINT ( 'NONE',  ( 33.07118982870879620, -279.8829693740426023, -295.8529559536213469 ) ) ;
#89559=CARTESIAN_POINT ( 'NONE',  ( 18.11967539104738023, -282.7756263267584700, -220.7088267491818669 ) ) ;
#89560=CARTESIAN_POINT ( 'NONE',  ( -110.1333905936174489, -270.7855059343972925, -253.8318528300186472 ) ) ;
#89561=CARTESIAN_POINT ( 'NONE',  ( -96.53789120484952946, -285.5017296358883527, -318.3633984162175921 ) ) ;
#89562=CARTESIAN_POINT ( 'NONE',  ( 34.30988347380085202, -286.6768228988213991, -285.9207998429771465 ) ) ;
#89563=CARTESIAN_POINT ( 'NONE',  ( 20.05813539071349538, -280.2058893438782547, -219.1693347566229022 ) ) ;
#89564=CARTESIAN_POINT ( 'NONE',  ( -38.02263352848247990, -140.5509088181942445, -364.3887990180761562 ) ) ;
#89566=CARTESIAN_POINT ( 'NONE',  ( 22.01124561654895828, -286.6234958640722539, -227.7398159755128404 ) ) ;
#89568=CARTESIAN_POINT ( 'NONE',  ( -104.1409881482590691, -285.1397499082257241, -308.1428741419522339 ) ) ;
#89569=CARTESIAN_POINT ( 'NONE',  ( 19.86942043269093006, -275.2449088329015581, -224.9651806263860294 ) ) ;
#89570=CARTESIAN_POINT ( 'NONE',  ( -47.68802408213801414, -290.8440142346942707, -194.3177641256785080 ) ) ;
#89571=CARTESIAN_POINT ( 'NONE',  ( 39.30944045300030609, -282.1264530914276634, -264.2035670107734973 ) ) ;
#89573=CARTESIAN_POINT ( 'NONE',  ( -113.5198228996071492, -280.1281459132346185, -265.9337754227978508 ) ) ;
#89574=CARTESIAN_POINT ( 'NONE',  ( 19.14176147960793273, -281.1727975640687873, -218.0604214638796350 ) ) ;
#89575=CARTESIAN_POINT ( 'NONE',  ( -102.0455923789670294, -281.6237833571633473, -301.4846348637937581 ) ) ;
#89576=CARTESIAN_POINT ( 'NONE',  ( -113.3214668634831810, -274.1400524880032208, -284.1914339370617881 ) ) ;
#89579=CARTESIAN_POINT ( 'NONE',  ( 26.96367716403861436, -278.0655883586620689, -308.6344360511462810 ) ) ;
#89580=CARTESIAN_POINT ( 'NONE',  ( 193.0921611339578305, 279.2154153515940607, -125.6430880757993549 ) ) ;
#89581=CARTESIAN_POINT ( 'NONE',  ( 35.05693201289778216, -279.3370976900665710, -252.1353739874853090 ) ) ;
#89582=CARTESIAN_POINT ( 'NONE',  ( -36.47356891843505622, -297.4118876466293386, -197.2592832589931788 ) ) ;
#89583=CARTESIAN_POINT ( 'NONE',  ( 32.17172918639448653, -293.4841391175193053, -303.4611917219432939 ) ) ;
#89585=CARTESIAN_POINT ( 'NONE',  ( -62.63277583733828635, -296.3040568366923253, -198.2572499750793042 ) ) ;
#89586=CARTESIAN_POINT ( 'NONE',  ( 21.80253129913998222, -286.5649270830892306, -314.5229525738844814 ) ) ;
#89587=CARTESIAN_POINT ( 'NONE',  ( 4.532336546358201268, -296.3408069062683126, -331.6590015584054072 ) ) ;
#89588=CARTESIAN_POINT ( 'NONE',  ( -42.72686556746183584, -287.2979985812592645, -197.0528173508388363 ) ) ;
#89589=CARTESIAN_POINT ( 'NONE',  ( 39.47615555355140060, -294.4926128789574591, -270.2981507593422634 ) ) ;
#89591=CARTESIAN_POINT ( 'NONE',  ( -102.2959638390236705, -285.4988446825265100, -236.9106760238458378 ) ) ;
#89592=CARTESIAN_POINT ( 'NONE',  ( -68.00434641705011529, -296.4535213656557744, -200.1062516053708009 ) ) ;
#89593=CARTESIAN_POINT ( 'NONE',  ( 22.97494117368558619, -293.7167107255746146, -222.7369285509479653 ) ) ;
#89594=CARTESIAN_POINT ( 'NONE',  ( -97.41944825924889528, -291.6888234764058438, -222.2966707987500570 ) ) ;
#89595=CARTESIAN_POINT ( 'NONE',  ( -80.40579356196042227, -289.8205086444457947, -329.3687714034125520 ) ) ;
#89598=CARTESIAN_POINT ( 'NONE',  ( 29.40725091552484116, -300.7397427917375126, -194.5754132039499211 ) ) ;
#89599=CARTESIAN_POINT ( 'NONE',  ( -105.2497983556404222, -271.8080301367127163, -234.7993882073907912 ) ) ;
#89601=CARTESIAN_POINT ( 'NONE',  ( 32.45191108217840537, -280.9060830272578642, -292.7131321126132661 ) ) ;
#89603=CARTESIAN_POINT ( 'NONE',  ( -22.95656013185844557, -276.3806422459417718, -345.9969674020971411 ) ) ;
#89604=CARTESIAN_POINT ( 'NONE',  ( -95.22765546882318688, -271.5910568669068539, -224.5827760291528534 ) ) ;
#89605=CARTESIAN_POINT ( 'NONE',  ( -104.4971973853501197, -280.8343585884473441, -238.6015539059482364 ) ) ;
#89606=CARTESIAN_POINT ( 'NONE',  ( 19.23467353355029630, -274.3638054465916412, -318.4233633109172388 ) ) ;
#89607=CARTESIAN_POINT ( 'NONE',  ( -100.2449718660991493, -298.2759484656190807, -232.4428217309732077 ) ) ;
#89608=CARTESIAN_POINT ( 'NONE',  ( -34.47848897105268406, -299.1684960680592553, -197.0514629679084919 ) ) ;
#89609=CARTESIAN_POINT ( 'NONE',  ( -101.6522597959774288, -298.6936015266034019, -229.4882378558616836 ) ) ;
#89610=CARTESIAN_POINT ( 'NONE',  ( -73.14075153709077881, -271.6005217377178838, -203.9944877908874616 ) ) ;
#89611=CARTESIAN_POINT ( 'NONE',  ( 14.94261957995175294, -293.4646942536728034, -219.1980916455273416 ) ) ;
#89612=CARTESIAN_POINT ( 'NONE',  ( 4.856258706341020748, -291.2090557548905281, -210.0101089810492567 ) ) ;
#89614=CARTESIAN_POINT ( 'NONE',  ( 39.07722661911996198, -276.1618146138142720, -279.7341719111043403 ) ) ;
#89615=CARTESIAN_POINT ( 'NONE',  ( -90.19806985006050581, -273.4451126151090534, -219.9920179780639273 ) ) ;
#89617=CARTESIAN_POINT ( 'NONE',  ( 25.51554251903686321, -280.8171480738862442, -313.9991184223015921 ) ) ;
#89620=CARTESIAN_POINT ( 'NONE',  ( -97.67128999651612276, -283.1734218353493020, -311.8371371473529621 ) ) ;
#89621=CARTESIAN_POINT ( 'NONE',  ( -112.0836631749813250, -282.4497652703412882, -278.3403024742773937 ) ) ;
#89622=CARTESIAN_POINT ( 'NONE',  ( 25.87252631797964852, -274.6407073834440666, -308.0352004666191306 ) ) ;
#89623=CARTESIAN_POINT ( 'NONE',  ( -0.5222142068229049805, -282.5415884900606898, -205.0065253237449099 ) ) ;
#89626=CARTESIAN_POINT ( 'NONE',  ( -7.979802776668437403, -272.8301804169730076, -199.9892464306108479 ) ) ;
#89627=CARTESIAN_POINT ( 'NONE',  ( -104.6911229971985904, -280.1114965826322418, -303.8560367657680672 ) ) ;
#89629=CARTESIAN_POINT ( 'NONE',  ( -112.3922429004825148, -286.5839443893443672, -261.6015388478689943 ) ) ;
#89631=CARTESIAN_POINT ( 'NONE',  ( -49.08822542786022325, -287.2015263728127366, -344.4875244724072445 ) ) ;
#89633=CARTESIAN_POINT ( 'NONE',  ( -101.5545765529196274, -295.8303392183124174, -234.8106326821514358 ) ) ;
#89634=CARTESIAN_POINT ( 'NONE',  ( -93.35914168139744618, -288.0081132860211710, -319.1505097427698843 ) ) ;
#89635=CARTESIAN_POINT ( 'NONE',  ( -110.2140734402150315, -271.0703965937372004, -283.6296548450457635 ) ) ;
#89636=CARTESIAN_POINT ( 'NONE',  ( -110.7310329344303312, -294.7512726589940826, -254.8396355759154233 ) ) ;
#89637=CARTESIAN_POINT ( 'NONE',  ( 24.99003905089042377, -285.4440322402592756, -226.3219713853931410 ) ) ;
#89638=CARTESIAN_POINT ( 'NONE',  ( 34.43292557344552307, -283.3770420041131501, -287.5859502710481479 ) ) ;
#89639=CARTESIAN_POINT ( 'NONE',  ( -94.58630382248043134, -282.1072233756623291, -320.3314027839390974 ) ) ;
#89640=CARTESIAN_POINT ( 'NONE',  ( -56.06559070839884384, -289.2999729422390942, -340.9715655669982652 ) ) ;
#89642=CARTESIAN_POINT ( 'NONE',  ( 26.96501145241477460, -282.4921625928938056, -234.5837262181236724 ) ) ;
#89643=CARTESIAN_POINT ( 'NONE',  ( -21.34296844787180092, -283.6446520213218037, -341.8040192261576635 ) ) ;
#89644=CARTESIAN_POINT ( 'NONE',  ( 34.27771780962692816, -289.2288727925524086, -246.7622623630037424 ) ) ;
#89646=CARTESIAN_POINT ( 'NONE',  ( -70.73096209601445139, -297.7905275210860054, -200.9769901882598333 ) ) ;
#89647=AXIS2_PLACEMENT_3D ( 'NONE', #92300, #57293, #43523 ) ;
#89648=CARTESIAN_POINT ( 'NONE',  ( -52.54562162856652208, -273.8627062079351617, -194.8226338173148235 ) ) ;
#89649=CARTESIAN_POINT ( 'NONE',  ( -69.75411472329601281, -293.6032317298727321, -203.1065217269365917 ) ) ;
#89651=CARTESIAN_POINT ( 'NONE',  ( -95.99890600148557951, -281.6948066931273615, -223.6242672951989618 ) ) ;
#89653=CARTESIAN_POINT ( 'NONE',  ( -6.071259384224857669, -274.6419973810752140, -338.7145229160199165 ) ) ;
#89655=CARTESIAN_POINT ( 'NONE',  ( -108.1376984480758807, -295.3149284291123990, -242.0349015764902560 ) ) ;
#89656=CARTESIAN_POINT ( 'NONE',  ( -104.7704509811376994, -291.7513341656749617, -300.4839769747057971 ) ) ;
#89657=CARTESIAN_POINT ( 'NONE',  ( -0.4877240763478836172, -273.9045122362478537, -207.2142865447675320 ) ) ;
#89659=CARTESIAN_POINT ( 'NONE',  ( -93.09359937935977314, -292.7524649219082562, -222.1694850611783920 ) ) ;
#89660=CARTESIAN_POINT ( 'NONE',  ( -65.42824781417573377, -292.6170040373164056, -202.7121077450888720 ) ) ;
#89661=CARTESIAN_POINT ( 'NONE',  ( -10.58885741231271815, -284.4586117343341698, -339.4245757958431113 ) ) ;
#89662=CARTESIAN_POINT ( 'NONE',  ( -69.39269039516942428, -293.0639061606021869, -200.9830593273178181 ) ) ;
#89663=CARTESIAN_POINT ( 'NONE',  ( -11.33672876627935189, -293.6990436908904485, -198.3537959456301678 ) ) ;
#89664=CARTESIAN_POINT ( 'NONE',  ( -18.22254538749057673, -294.6321011485756003, -340.8129307803160941 ) ) ;
#89665=CARTESIAN_POINT ( 'NONE',  ( 28.10039044746680048, -289.0632564918700496, -233.6170537162354606 ) ) ;
#89666=CARTESIAN_POINT ( 'NONE',  ( 38.79440189358674473, -281.5706601735786876, -258.5134536059317156 ) ) ;
#89667=CARTESIAN_POINT ( 'NONE',  ( -109.8480107706053275, -270.9742156050767221, -248.2015136030119606 ) ) ;
#89668=CARTESIAN_POINT ( 'NONE',  ( -93.91829464007776096, -285.0973030077281010, -218.0518669750361482 ) ) ;
#89670=CARTESIAN_POINT ( 'NONE',  ( 19.57864721398203045, -278.2034925973981103, -318.6510844766171999 ) ) ;
#89672=CARTESIAN_POINT ( 'NONE',  ( -8.098805183234398797, -284.4348554765707036, -201.2417963333080877 ) ) ;
#89673=CARTESIAN_POINT ( 'NONE',  ( -96.97166545007570448, -276.0567778406275465, -317.1005309045386298 ) ) ;
#89675=CARTESIAN_POINT ( 'NONE',  ( -42.94388623651373393, -282.6322750248692159, -343.2576875936265992 ) ) ;
#89677=CARTESIAN_POINT ( 'NONE',  ( -71.07364184738068502, -280.8218972447962756, -201.5849242211563705 ) ) ;
#89678=CARTESIAN_POINT ( 'NONE',  ( 39.36856562693941441, -286.6618503214559155, -274.4224749626239372 ) ) ;
#89679=CARTESIAN_POINT ( 'NONE',  ( 19.62723108426097340, -295.9732243509820933, -317.6106141975219543 ) ) ;
#89680=CARTESIAN_POINT ( 'NONE',  ( 34.45414767977475634, -277.4796374117198070, -296.0470743823016733 ) ) ;
#89681=CARTESIAN_POINT ( 'NONE',  ( 9.197014594869811432, -275.9916088280801318, -209.6367711077459148 ) ) ;
#89682=CARTESIAN_POINT ( 'NONE',  ( -109.6215042494474829, -278.5250331579922545, -259.7815659572450500 ) ) ;
#89683=CARTESIAN_POINT ( 'NONE',  ( -107.8685235036640222, -274.8500381991245263, -245.9108830901979559 ) ) ;
#89684=CARTESIAN_POINT ( 'NONE',  ( -7.501052274080759474, -284.4441422001780211, -201.7348535889083507 ) ) ;
#89685=CARTESIAN_POINT ( 'NONE',  ( -101.6153986926417758, -291.6089879079249272, -311.3889997558484311 ) ) ;
#89687=CARTESIAN_POINT ( 'NONE',  ( 27.76735225481852254, -292.0162625881526424, -236.6708023046132325 ) ) ;
#89689=CARTESIAN_POINT ( 'NONE',  ( -64.07540055819274016, -291.3603113067068762, -202.3961520365329534 ) ) ;
#89691=CARTESIAN_POINT ( 'NONE',  ( -15.02899007471783044, -289.8495555660354057, -343.7899098780044937 ) ) ;
#89692=CARTESIAN_POINT ( 'NONE',  ( -72.18558837658798666, -280.2296655386205089, -206.0976281915633592 ) ) ;
#89693=CARTESIAN_POINT ( 'NONE',  ( -91.40782768564372418, -296.2246694600536330, -215.9704353222274449 ) ) ;
#89694=CARTESIAN_POINT ( 'NONE',  ( 14.54106201777362628, -288.9964586877092643, -327.1914694694860941 ) ) ;
#89696=CARTESIAN_POINT ( 'NONE',  ( 38.76402612248147506, -287.7397053376743656, -258.7121262874467789 ) ) ;
#89697=CARTESIAN_POINT ( 'NONE',  ( -98.12701881504915491, -285.4469649222994576, -229.8983879844416265 ) ) ;
#89698=CARTESIAN_POINT ( 'NONE',  ( -22.45178514855419749, -108.0970913119723633, -362.6615123362100803 ) ) ;
#89699=CARTESIAN_POINT ( 'NONE',  ( 119.9967176495213721, 149.6214322644071046, -262.1809137269642633 ) ) ;
#89700=CARTESIAN_POINT ( 'NONE',  ( 166.9733864952704323, 230.1165055869454079, -189.8826931914318834 ) ) ;
#89701=CARTESIAN_POINT ( 'NONE',  ( -13.74296406813424554, -275.9351860388663908, -339.6653729485777262 ) ) ;
#89702=CARTESIAN_POINT ( 'NONE',  ( -87.31625309304148175, -276.6892941211253287, -323.9966484537966380 ) ) ;
#89703=CARTESIAN_POINT ( 'NONE',  ( -111.7967352951812217, -272.4659885200412077, -250.6074206108544615 ) ) ;
#89704=CARTESIAN_POINT ( 'NONE',  ( 154.7032878266783484, 204.3872195088065098, -214.8778263170268588 ) ) ;
#89705=CARTESIAN_POINT ( 'NONE',  ( -64.93295899708127195, -276.0898287494861165, -341.7754456001293306 ) ) ;
#89707=CARTESIAN_POINT ( 'NONE',  ( -39.95393263892906077, -289.5780757828688365, -343.4255622367987826 ) ) ;
#89708=CARTESIAN_POINT ( 'NONE',  ( -98.96906488981969119, -297.9668980725343204, -224.4455086316405357 ) ) ;
#89709=CARTESIAN_POINT ( 'NONE',  ( -109.3777085860852338, -296.7006794720535368, -297.5362061286186872 ) ) ;
#89710=CARTESIAN_POINT ( 'NONE',  ( 3.818136636171794773, -294.6473437734380809, -330.6509831510050503 ) ) ;
#89713=CARTESIAN_POINT ( 'NONE',  ( -79.40389585043679688, -279.5349971063639032, -333.1941933107227669 ) ) ;
#89715=CARTESIAN_POINT ( 'NONE',  ( 11.44873081016254091, -281.9042857687664423, -329.9197245529882139 ) ) ;
#89718=CARTESIAN_POINT ( 'NONE',  ( -107.5270165688972952, -279.9109494194071885, -249.1892633164697202 ) ) ;
#89719=CARTESIAN_POINT ( 'NONE',  ( 32.10288438361173746, -277.7112051631133340, -301.2062747073114224 ) ) ;
#89720=CARTESIAN_POINT ( 'NONE',  ( -86.48037005042883152, -295.9282185874638458, -215.5818697765060961 ) ) ;
#89722=CARTESIAN_POINT ( 'NONE',  ( -83.00510463768449654, -277.8636661250710063, -327.3810119664037757 ) ) ;
#89724=CARTESIAN_POINT ( 'NONE',  ( 7.133180848106611904, -275.4434979990307966, -207.6368785608249539 ) ) ;
#89725=CARTESIAN_POINT ( 'NONE',  ( 5.268687897342505089, -287.1734711991509243, -333.9036478670230395 ) ) ;
#89726=CARTESIAN_POINT ( 'NONE',  ( -3.483820065667599497, -276.4991874008418904, -203.4241227442792308 ) ) ;
#89727=CARTESIAN_POINT ( 'NONE',  ( 34.63973520401290074, -274.4547242220602925, -296.1544280080917702 ) ) ;
#89729=CIRCLE ( 'NONE', #49007, 2.500000000000008882 ) ;
#89730=CARTESIAN_POINT ( 'NONE',  ( -94.23629677755644707, -289.1001973245907379, -316.3568416929266505 ) ) ;
#89732=CARTESIAN_POINT ( 'NONE',  ( -111.0127099063557523, -283.6232389378021139, -292.4498882909786630 ) ) ;
#89733=CARTESIAN_POINT ( 'NONE',  ( 32.30057180541375317, -280.1229499570794701, -295.5710139224876798 ) ) ;
#89734=CARTESIAN_POINT ( 'NONE',  ( 28.67167796277082914, -280.5654193931208624, -302.9976018816071814 ) ) ;
#89735=CARTESIAN_POINT ( 'NONE',  ( -110.0665815853239025, -282.8382930184193924, -254.4144102647672412 ) ) ;
#89736=CARTESIAN_POINT ( 'NONE',  ( -42.15725490279448451, -291.1129995634192937, -345.2191098186257250 ) ) ;
#89737=CARTESIAN_POINT ( 'NONE',  ( -72.33244455524882710, -280.7832386031947749, -205.8415216573589532 ) ) ;
#89739=CARTESIAN_POINT ( 'NONE',  ( -64.98120794621493701, -281.8071227091404012, -341.3857245747802835 ) ) ;
#89740=CARTESIAN_POINT ( 'NONE',  ( 18.06970972713684631, -296.2584298839960866, -320.9796108451695886 ) ) ;
#89742=CARTESIAN_POINT ( 'NONE',  ( -81.62983120171526252, -277.6982242743594611, -208.6153856801973348 ) ) ;
#89743=CARTESIAN_POINT ( 'NONE',  ( -101.9431346154957936, -278.7381712298223420, -304.5743804698732333 ) ) ;
#89744=CARTESIAN_POINT ( 'NONE',  ( -44.22533246178981159, -285.1390435861054016, -345.2640160457759748 ) ) ;
#89746=CARTESIAN_POINT ( 'NONE',  ( -109.8572015051091029, -292.7436878732109449, -249.1286838525142855 ) ) ;
#89747=AXIS2_PLACEMENT_3D ( 'NONE', #62456, #91299, #19818 ) ;
#89748=CARTESIAN_POINT ( 'NONE',  ( -70.34881503073090414, -271.6169354810726304, -203.0147667888204239 ) ) ;
#89749=CARTESIAN_POINT ( 'NONE',  ( 37.22261248932176869, -286.5166871011144849, -251.8051996535899377 ) ) ;
#89750=CARTESIAN_POINT ( 'NONE',  ( -110.7668025937934289, -289.0489600255833125, -262.9318015864479889 ) ) ;
#89752=CARTESIAN_POINT ( 'NONE',  ( -8.560885869508723545, -275.3522351774336130, -337.9980318598725830 ) ) ;
#89753=CARTESIAN_POINT ( 'NONE',  ( -31.52887850723255880, -293.1177069419536565, -344.4193532260970301 ) ) ;
#89755=CARTESIAN_POINT ( 'NONE',  ( -3.610238903460962323, -290.9690894537313852, -201.9004068496637672 ) ) ;
#89756=CARTESIAN_POINT ( 'NONE',  ( -108.1280509493019650, -286.4275845287461379, -249.3094907452707218 ) ) ;
#89757=CARTESIAN_POINT ( 'NONE',  ( 7.320561967526738378, -286.6928955798195489, -331.9016473640056688 ) ) ;
#89758=CARTESIAN_POINT ( 'NONE',  ( 35.14461996519094100, -288.8075732341791877, -257.3812306982285349 ) ) ;
#89760=CARTESIAN_POINT ( 'NONE',  ( 17.95427823071062079, -289.0368565060061883, -318.3426870941156608 ) ) ;
#89761=CARTESIAN_POINT ( 'NONE',  ( 36.44606664042736810, -295.3358420602150431, -255.0083620571739687 ) ) ;
#89763=CARTESIAN_POINT ( 'NONE',  ( 36.98780169253481631, -288.5242705936230436, -251.8372447611259020 ) ) ;
#89764=CARTESIAN_POINT ( 'NONE',  ( -35.76651257513341875, -275.1124205830040523, -345.9175797689611045 ) ) ;
#89765=CARTESIAN_POINT ( 'NONE',  ( -56.91455420214910532, -277.6310357544087992, -344.8651147841035822 ) ) ;
#89766=CARTESIAN_POINT ( 'NONE',  ( -63.86008293881810260, -289.7890288565636752, -199.5522787797956141 ) ) ;
#89767=CARTESIAN_POINT ( 'NONE',  ( -68.66003520145358152, -279.3184128645539772, -200.0267097626730219 ) ) ;
#89768=CARTESIAN_POINT ( 'NONE',  ( -34.42409459764055413, -300.0687386000333277, -195.7153189856822735 ) ) ;
#89770=CARTESIAN_POINT ( 'NONE',  ( -105.2868320042121297, -282.9708252739504246, -238.4818388863222935 ) ) ;
#89772=CARTESIAN_POINT ( 'NONE',  ( -97.10120406042616992, -276.0845272991123807, -314.4240863681287124 ) ) ;
#89773=CARTESIAN_POINT ( 'NONE',  ( 35.06112930142459305, -279.2998677739368532, -250.7462862747766223 ) ) ;
#89774=CARTESIAN_POINT ( 'NONE',  ( -53.99892735073297700, -275.7419907114563671, -344.8816677552685519 ) ) ;
#89775=CARTESIAN_POINT ( 'NONE',  ( -109.7303514691843418, -298.2535604188194611, -256.4883524508573487 ) ) ;
#89776=CARTESIAN_POINT ( 'NONE',  ( 22.27426092079513609, -281.1222233881068746, -318.6252747122812821 ) ) ;
#89777=CARTESIAN_POINT ( 'NONE',  ( -94.64289221352605352, -298.1353674368834845, -224.7543001308467012 ) ) ;
#89778=CARTESIAN_POINT ( 'NONE',  ( -111.1508008949219573, -298.1233897627992064, -250.0277956969105162 ) ) ;
#89779=CARTESIAN_POINT ( 'NONE',  ( 19.01787927376628673, -274.5610674547732515, -223.9317598509602476 ) ) ;
#89780=CARTESIAN_POINT ( 'NONE',  ( 32.68696770348992686, -295.2032517795659601, -243.5099293965219545 ) ) ;
#89781=CARTESIAN_POINT ( 'NONE',  ( 23.86014298253209986, -287.0956129528201473, -223.6133365455938815 ) ) ;
#89782=CARTESIAN_POINT ( 'NONE',  ( -47.89304872393783086, -277.9989449497981582, -195.4886110040247331 ) ) ;
#89783=CARTESIAN_POINT ( 'NONE',  ( -99.20332520864903358, -290.9952337031335219, -224.4899379185518740 ) ) ;
#89785=CARTESIAN_POINT ( 'NONE',  ( 13.31092110019945629, -285.8402695796268063, -217.3976598597944871 ) ) ;
#89786=CARTESIAN_POINT ( 'NONE',  ( -112.3891538888654793, -288.5414624955303680, -271.1808003295139997 ) ) ;
#89790=CARTESIAN_POINT ( 'NONE',  ( 34.34331779029790255, -287.2467051061422580, -284.5412388223898574 ) ) ;
#89792=CARTESIAN_POINT ( 'NONE',  ( -96.08250420123283675, -284.8256802426582226, -319.8014701400959439 ) ) ;
#89793=CARTESIAN_POINT ( 'NONE',  ( 36.85824857785865305, -292.3632274944400251, -250.6332838989275160 ) ) ;
#89794=CARTESIAN_POINT ( 'NONE',  ( 31.29195311423949022, -282.7217399448792321, -237.1359866008581605 ) ) ;
#89795=CARTESIAN_POINT ( 'NONE',  ( 16.86182612839302664, -282.1192778667672769, -216.2935534489989493 ) ) ;
#89797=CARTESIAN_POINT ( 'NONE',  ( -66.56152234411779034, -283.2791404369732504, -337.2716397958188850 ) ) ;
#89798=CARTESIAN_POINT ( 'NONE',  ( -99.92155132198499246, -297.1466648004941931, -225.4972993248834712 ) ) ;
#89800=CARTESIAN_POINT ( 'NONE',  ( -107.6733376637402415, -274.1498483899442249, -248.8628631591116118 ) ) ;
#89801=CARTESIAN_POINT ( 'NONE',  ( -38.90735864321626281, -290.0525215615998036, -195.7327351814898009 ) ) ;
#89802=CARTESIAN_POINT ( 'NONE',  ( -96.59287825623330548, -271.9514021800117121, -226.9589390155948649 ) ) ;
#89805=CARTESIAN_POINT ( 'NONE',  ( -109.7722178267710120, -286.6952035556068381, -253.1266692692933304 ) ) ;
#89807=CARTESIAN_POINT ( 'NONE',  ( -66.79297008120266810, -296.5087523345606542, -341.1856787204346233 ) ) ;
#89809=CARTESIAN_POINT ( 'NONE',  ( -109.5231000566148509, -285.3569559644520837, -258.7172503771982406 ) ) ;
#89810=CARTESIAN_POINT ( 'NONE',  ( -31.48023023705274426, -276.0387371632383520, -346.9541801191982131 ) ) ;
#89811=CARTESIAN_POINT ( 'NONE',  ( -8.557082626845954110, -293.0705725152864147, -199.0536248140858220 ) ) ;
#89812=CARTESIAN_POINT ( 'NONE',  ( 4.517305946693795704, -284.7496038322475442, -207.1469824801062884 ) ) ;
#89813=CARTESIAN_POINT ( 'NONE',  ( -50.56689613274777884, -292.2209497488270813, -194.5268349564630626 ) ) ;
#89814=CARTESIAN_POINT ( 'NONE',  ( -107.7450554036466031, -290.6272667590225751, -289.9240742387481191 ) ) ;
#89818=CARTESIAN_POINT ( 'NONE',  ( -54.88761368322284540, -169.8575745514222035, -360.7447470472093300 ) ) ;
#89819=CARTESIAN_POINT ( 'NONE',  ( -98.79746901162829431, -286.6796149700505794, -225.0425659211572054 ) ) ;
#89820=CARTESIAN_POINT ( 'NONE',  ( 36.60358173371529489, -272.6237833571633473, -234.7871824221999191 ) ) ;
#89822=CARTESIAN_POINT ( 'NONE',  ( -34.84974809406566010, -281.9404765767924914, -343.6403546193134844 ) ) ;
#89823=CARTESIAN_POINT ( 'NONE',  ( -74.09049100538294397, -277.1934562704336145, -338.0168632654421685 ) ) ;
#89824=CARTESIAN_POINT ( 'NONE',  ( -41.16981823186733180, -282.0040053090052652, -195.6257586131330584 ) ) ;
#89825=CARTESIAN_POINT ( 'NONE',  ( 27.39393885966332576, -24.46849793231620396, -343.6547034384808512 ) ) ;
#89826=CARTESIAN_POINT ( 'NONE',  ( -19.07696777372116159, -281.3964061385267996, -344.6113786719984660 ) ) ;
#89827=CARTESIAN_POINT ( 'NONE',  ( 34.62154628106470255, -285.3160390568893376, -250.5334108281160184 ) ) ;
#89828=CARTESIAN_POINT ( 'NONE',  ( -37.27724884726870158, -299.8130847980922908, -194.3736719644936102 ) ) ;
#89830=CARTESIAN_POINT ( 'NONE',  ( -18.19834555420284161, -295.2910223096777145, -340.8701274574840454 ) ) ;
#89832=CARTESIAN_POINT ( 'NONE',  ( -14.67852482912937440, -291.0369281710678138, -200.4495741389052057 ) ) ;
#89833=CARTESIAN_POINT ( 'NONE',  ( -101.8102993582165681, -279.7558828500485788, -228.3468240315060598 ) ) ;
#89834=CARTESIAN_POINT ( 'NONE',  ( -4.104686705431316973, -274.5031169435301308, -205.3524627330299097 ) ) ;
#89835=CARTESIAN_POINT ( 'NONE',  ( 37.60066400795967922, -274.6777176620538512, -286.7053776213849119 ) ) ;
#89837=CARTESIAN_POINT ( 'NONE',  ( -52.72996239112953276, -271.8549484850714180, -196.9042698117588941 ) ) ;
#89838=CARTESIAN_POINT ( 'NONE',  ( -16.64886731540296338, -296.2153200427665070, -343.9714416967875081 ) ) ;
#89841=CARTESIAN_POINT ( 'NONE',  ( -61.62419700654685073, -284.4547478530649869, -339.5852801861693706 ) ) ;
#89842=CARTESIAN_POINT ( 'NONE',  ( 4.013252073238731121, -284.2638766398117127, -334.1708030930938094 ) ) ;
#89843=CARTESIAN_POINT ( 'NONE',  ( -96.65267670545426881, -284.4977436308168421, -227.6068667201013511 ) ) ;
#89844=CARTESIAN_POINT ( 'NONE',  ( -36.47702481675179342, -275.4410438882899825, -344.1686593674873507 ) ) ;
#89845=CARTESIAN_POINT ( 'NONE',  ( -40.25958646312011524, -284.9496379451209123, -344.5389544407888138 ) ) ;
#89846=CARTESIAN_POINT ( 'NONE',  ( -35.11590675149710705, -275.5035730322827590, -344.0208328738047499 ) ) ;
#89847=CARTESIAN_POINT ( 'NONE',  ( -8.863391098975974103, -275.5132116173144823, -202.7554329741854815 ) ) ;
#89849=CARTESIAN_POINT ( 'NONE',  ( -67.30893073698736373, -280.4718600113618550, -199.6071505291407959 ) ) ;
#89853=CARTESIAN_POINT ( 'NONE',  ( 38.46692529297811802, -289.4271534675118005, -271.5085520155910217 ) ) ;
#89854=CARTESIAN_POINT ( 'NONE',  ( -34.30470247405479256, -294.2101596997219985, -343.4595336464529964 ) ) ;
#89856=CARTESIAN_POINT ( 'NONE',  ( -111.8253781160310041, -289.6605803078348913, -289.5317281382592682 ) ) ;
#89857=CARTESIAN_POINT ( 'NONE',  ( -4.119895180196953000, -284.7362822176437476, -204.2227350859878072 ) ) ;
#89858=CARTESIAN_POINT ( 'NONE',  ( 33.96398600394710598, -285.8881044716035831, -252.1202626243413363 ) ) ;
#89859=CARTESIAN_POINT ( 'NONE',  ( -80.09807245662983632, -289.7048138470740923, -209.8841849596891223 ) ) ;
#89860=CARTESIAN_POINT ( 'NONE',  ( -8.110837002141366270, -287.6488603328508589, -203.0358838827385455 ) ) ;
#89861=CARTESIAN_POINT ( 'NONE',  ( -81.39271181780156894, -275.6511190905586659, -331.0612746139123601 ) ) ;
#89862=CARTESIAN_POINT ( 'NONE',  ( 37.32031443120019532, -286.1445309829779262, -285.5934520003472699 ) ) ;
#89863=CARTESIAN_POINT ( 'NONE',  ( -36.61118143951127024, -288.0614788422674337, -195.3519716531124004 ) ) ;
#89864=CARTESIAN_POINT ( 'NONE',  ( 33.14412335963569234, -285.2138356135331492, -244.2502560263469036 ) ) ;
#89865=CARTESIAN_POINT ( 'NONE',  ( 35.80151961470608057, -282.5416835992856477, -274.0323375544222131 ) ) ;
#89866=CARTESIAN_POINT ( 'NONE',  ( 20.99872652587955102, -290.2038471282730256, -317.7778294364557610 ) ) ;
#89867=CARTESIAN_POINT ( 'NONE',  ( 83.14890176555634582, -299.5541904835127980, -197.2570935515975918 ) ) ;
#89869=CARTESIAN_POINT ( 'NONE',  ( -109.4464886090978837, -298.7635182668197444, -247.5995829736514793 ) ) ;
#89870=CARTESIAN_POINT ( 'NONE',  ( 36.18652026696772595, -279.7426621459921989, -285.2108185068661328 ) ) ;
#89871=CARTESIAN_POINT ( 'NONE',  ( -34.95516457603115867, -291.2785498861794622, -193.5465420314574203 ) ) ;
#89872=CARTESIAN_POINT ( 'NONE',  ( -110.5268743519827410, -295.0810902075823492, -260.4695318092544198 ) ) ;
#89873=CARTESIAN_POINT ( 'NONE',  ( 3.651497655673336951, -281.1730013320150192, -331.4210378835179540 ) ) ;
#89874=CARTESIAN_POINT ( 'NONE',  ( 32.47723748092739982, -273.2943781902573619, -244.5419362090048878 ) ) ;
#89875=CARTESIAN_POINT ( 'NONE',  ( -95.15104289980627073, -297.2316850054183988, -315.7408862491202513 ) ) ;
#89877=CARTESIAN_POINT ( 'NONE',  ( -20.67871297045058654, -296.7370723534652939, -194.0586629801171341 ) ) ;
#89878=CARTESIAN_POINT ( 'NONE',  ( 25.65889246766253962, -292.3592539969980635, -312.8452249672719745 ) ) ;
#89881=CARTESIAN_POINT ( 'NONE',  ( 33.27524152560594217, -294.6076599488613965, -289.5359632295803181 ) ) ;
#89883=CARTESIAN_POINT ( 'NONE',  ( -47.06954514272372592, -281.1952504626975156, -345.0857848100808383 ) ) ;
#89884=CARTESIAN_POINT ( 'NONE',  ( 17.97243039637194428, -294.2307742803172346, -318.0178407332722941 ) ) ;
#89885=CARTESIAN_POINT ( 'NONE',  ( -13.42193596962568414, -282.7499011540667198, -343.5515878717734495 ) ) ;
#89886=CARTESIAN_POINT ( 'NONE',  ( 14.16158275542191447, -282.6884595793933954, -215.0019489326299720 ) ) ;
#89887=CARTESIAN_POINT ( 'NONE',  ( -54.95564823339118732, -285.4983639566385705, -195.4245239608235067 ) ) ;
#89889=CARTESIAN_POINT ( 'NONE',  ( -110.9875841250319723, -288.3811207866403947, -283.6393783691144108 ) ) ;
#89890=CARTESIAN_POINT ( 'NONE',  ( 38.11214887289218467, -279.8841303986320099, -258.6413628431546954 ) ) ;
#89892=CARTESIAN_POINT ( 'NONE',  ( -12.33755586500258339, -287.6548295491841145, -342.9170043981440017 ) ) ;
#89894=CARTESIAN_POINT ( 'NONE',  ( -5.174593117775942552, -296.2216817528400838, -336.7958443613134705 ) ) ;
#89895=CARTESIAN_POINT ( 'NONE',  ( -62.19703594111321365, -278.7943127760404991, -342.6722225098698118 ) ) ;
#89896=CARTESIAN_POINT ( 'NONE',  ( 37.80279614241336361, -291.5002937487391819, -264.7298232078958335 ) ) ;
#89897=CARTESIAN_POINT ( 'NONE',  ( -91.30958548241221706, -278.9240228655258989, -221.1721472961937707 ) ) ;
#89898=CARTESIAN_POINT ( 'NONE',  ( 8.849230703342058746, -292.8324343640053939, -208.6877723966226768 ) ) ;
#89899=CARTESIAN_POINT ( 'NONE',  ( -111.7239106847011811, -282.4589670732569289, -283.9380352956530373 ) ) ;
#89900=CARTESIAN_POINT ( 'NONE',  ( -74.32716041703696419, -279.5441218682748854, -335.6073927946701474 ) ) ;
#89901=CARTESIAN_POINT ( 'NONE',  ( 23.54350313674527584, -292.0475267887983364, -229.6622178550532567 ) ) ;
#89902=CARTESIAN_POINT ( 'NONE',  ( -95.50094917528325311, -271.2071589797232605, -222.7224496431605587 ) ) ;
#89905=CARTESIAN_POINT ( 'NONE',  ( 1.597331475843968507, -294.0242067541956317, -332.2412583215452742 ) ) ;
#89907=CARTESIAN_POINT ( 'NONE',  ( -21.39648532958014826, -286.3380690714489560, -340.3683826091709079 ) ) ;
#89908=CARTESIAN_POINT ( 'NONE',  ( -82.82150239962889771, -296.5061975434459214, -208.4532835692209005 ) ) ;
#89911=CARTESIAN_POINT ( 'NONE',  ( -33.76723103276980709, -287.4114192802107368, -193.9378136556935033 ) ) ;
#89912=CARTESIAN_POINT ( 'NONE',  ( 14.08187707290968049, -288.1384062289997701, -322.1743953576719832 ) ) ;
#89913=CARTESIAN_POINT ( 'NONE',  ( -101.1738028703902046, -279.5708470231476213, -307.2897784851741676 ) ) ;
#89914=CARTESIAN_POINT ( 'NONE',  ( -75.75548366577658044, -299.2923768206337058, -207.0375180098544092 ) ) ;
#89915=CARTESIAN_POINT ( 'NONE',  ( -98.31495743973337653, -277.9125917595251849, -229.4126990596184612 ) ) ;
#89916=VERTEX_POINT ( 'NONE', #49103 ) ;
#89917=CARTESIAN_POINT ( 'NONE',  ( -91.61761176654559335, -296.9709393805669606, -215.7729351286436383 ) ) ;
#89918=CARTESIAN_POINT ( 'NONE',  ( -85.60033671758756668, -291.6455633707108177, -327.1073345188580674 ) ) ;
#89919=CARTESIAN_POINT ( 'NONE',  ( 31.45483283253144791, -294.7264885315386778, -237.4745970609529309 ) ) ;
#89921=CARTESIAN_POINT ( 'NONE',  ( -97.42796936618576353, -290.6240069292109638, -312.0188232723045871 ) ) ;
#89923=CARTESIAN_POINT ( 'NONE',  ( -5.107791317458369562, -290.6115325695580509, -201.7952328262568642 ) ) ;
#89924=CARTESIAN_POINT ( 'NONE',  ( -99.07802444478326720, -297.4974225790109017, -224.3568313837498636 ) ) ;
#89925=CARTESIAN_POINT ( 'NONE',  ( -96.89752427075154628, -296.8086887944205046, -228.1095937792574944 ) ) ;
#89927=CARTESIAN_POINT ( 'NONE',  ( 82.64890176555634582, -299.5541904835127980, -195.3611179825600175 ) ) ;
#89928=CARTESIAN_POINT ( 'NONE',  ( -96.73807863619954617, -291.4240148852437642, -318.2855591002485767 ) ) ;
#89929=CARTESIAN_POINT ( 'NONE',  ( -115.3430155898818299, -293.2662352645559167, -252.5904736702033517 ) ) ;
#89930=CARTESIAN_POINT ( 'NONE',  ( 26.50187938659362530, -289.0275910420738796, -231.3223452077258457 ) ) ;
#89931=CARTESIAN_POINT ( 'NONE',  ( 32.84646208357424513, -273.2143846631282713, -244.4063436589451612 ) ) ;
#89932=CARTESIAN_POINT ( 'NONE',  ( 21.16921154658293602, -278.1090717182042908, -316.4010783418359551 ) ) ;
#89933=CARTESIAN_POINT ( 'NONE',  ( -32.03061151134350126, -290.1994883993817211, -196.0979521634439209 ) ) ;
#89934=CARTESIAN_POINT ( 'NONE',  ( -79.51858870759124898, -279.4752685990683858, -333.3640381407938094 ) ) ;
#89936=CARTESIAN_POINT ( 'NONE',  ( 17.67611166433070480, -281.5865838464993658, -318.4956487684563058 ) ) ;
#89937=CARTESIAN_POINT ( 'NONE',  ( -97.67717078006829468, -278.9963892631488989, -317.7016238148365233 ) ) ;
#89938=CARTESIAN_POINT ( 'NONE',  ( 27.52334373093404807, -279.8096424740933799, -229.5120189446091388 ) ) ;
#89940=CARTESIAN_POINT ( 'NONE',  ( -113.1080972910931024, -270.6751398228194034, -270.3372191192045761 ) ) ;
#89941=CARTESIAN_POINT ( 'NONE',  ( 38.68947411932053626, -276.3605926166272297, -259.7742980904465639 ) ) ;
#89942=CARTESIAN_POINT ( 'NONE',  ( -27.10883676588594682, -275.6999603168554813, -194.6907365096304829 ) ) ;
#89943=CARTESIAN_POINT ( 'NONE',  ( 31.03373250439201669, -301.4082689599840705, -195.3320873922940848 ) ) ;
#89947=DIRECTION ( 'NONE',  ( -1.000000000000000000, -0.000000000000000000, -0.000000000000000000 ) ) ;
#89948=CARTESIAN_POINT ( 'NONE',  ( -50.79475610227913762, -290.3076064726240588, -342.4771613618003698 ) ) ;
#89949=CARTESIAN_POINT ( 'NONE',  ( -99.83429374786048527, -291.7337639988218712, -313.5889996891918940 ) ) ;
#89950=CARTESIAN_POINT ( 'NONE',  ( -109.0403350769879012, -289.7121110847018599, -284.6799490144572360 ) ) ;
#89951=CARTESIAN_POINT ( 'NONE',  ( 30.08065940350859435, -286.5781675359449991, -233.1863923119585706 ) ) ;
#89953=CARTESIAN_POINT ( 'NONE',  ( 35.26893285779855347, -280.1251340339272815, -283.6278980665212543 ) ) ;
#89954=CARTESIAN_POINT ( 'NONE',  ( -18.13139690053984054, -290.6624792496601799, -342.1211510195499272 ) ) ;
#89955=CARTESIAN_POINT ( 'NONE',  ( -13.32149529327954340, -281.2144630202237749, -340.0839961675785617 ) ) ;
#89956=CARTESIAN_POINT ( 'NONE',  ( 30.47012436447508676, -282.4897937925332485, -242.0273936280131011 ) ) ;
#89957=CARTESIAN_POINT ( 'NONE',  ( -4.423062348311134429, -289.5701354822533062, -339.7238313491587292 ) ) ;
#89958=CARTESIAN_POINT ( 'NONE',  ( -106.3202312655517687, -278.7226032226615189, -294.5966783749041156 ) ) ;
#89959=CARTESIAN_POINT ( 'NONE',  ( -111.9271295817409708, -289.5666440736679874, -252.8962265219410028 ) ) ;
#89961=CARTESIAN_POINT ( 'NONE',  ( -97.46046614397103269, -285.9969746689826593, -222.5082936754134266 ) ) ;
#89962=CARTESIAN_POINT ( 'NONE',  ( -83.24419353751396500, -285.9348222748192825, -208.5493295224553378 ) ) ;
#89963=CARTESIAN_POINT ( 'NONE',  ( -73.79495122221321424, -283.7169860311362299, -333.6655429074372137 ) ) ;
#89966=CARTESIAN_POINT ( 'NONE',  ( -63.97711796632140846, -293.5689891483524434, -199.3772824239310637 ) ) ;
#89967=CARTESIAN_POINT ( 'NONE',  ( -3.462327495357582663, -293.2991735245171299, -338.9721750415013730 ) ) ;
#89968=CARTESIAN_POINT ( 'NONE',  ( -76.49169910805632355, -276.6483234226089962, -332.3133016373562896 ) ) ;
#89969=CARTESIAN_POINT ( 'NONE',  ( -112.2084711431010646, -295.6801526898366319, -287.9759849426580445 ) ) ;
#89970=CARTESIAN_POINT ( 'NONE',  ( -25.27669040141606871, -290.6884702498393835, -197.6101573193406580 ) ) ;
#89971=CARTESIAN_POINT ( 'NONE',  ( -6.360878613344971733, -292.8793467238133417, -337.5783978623062467 ) ) ;
#89972=CARTESIAN_POINT ( 'NONE',  ( -30.78671084144532699, -293.3419363980237335, -197.2573381877226382 ) ) ;
#89974=CARTESIAN_POINT ( 'NONE',  ( 16.20199196301189204, -290.8091783406275681, -217.5326901332017826 ) ) ;
#89975=CARTESIAN_POINT ( 'NONE',  ( 36.63390184229079694, -295.3898195050147706, -257.7057802422615396 ) ) ;
#89976=CARTESIAN_POINT ( 'NONE',  ( 31.62499701618000358, -288.8203895685710449, -294.9985515516568739 ) ) ;
#89977=CARTESIAN_POINT ( 'NONE',  ( -35.72105268046706072, -279.0118359600550093, -345.7117356905076804 ) ) ;
#89978=CARTESIAN_POINT ( 'NONE',  ( -68.86606538362335073, -276.2523913870165870, -340.1910864744706942 ) ) ;
#89979=CARTESIAN_POINT ( 'NONE',  ( -48.93550933732409192, -297.1053589863586808, -194.3487443504060650 ) ) ;
#89980=CARTESIAN_POINT ( 'NONE',  ( -66.61387008749871086, -277.7455892132325062, -201.9041390836186167 ) ) ;
#89981=CARTESIAN_POINT ( 'NONE',  ( -98.17716941829219479, -276.3343318637661810, -316.2681162950927956 ) ) ;
#89982=CARTESIAN_POINT ( 'NONE',  ( -110.5922315924300534, -295.1509359700516484, -276.9271489052590596 ) ) ;
#89984=CARTESIAN_POINT ( 'NONE',  ( -110.4439418194319558, -273.2393927828638311, -267.6417298770065827 ) ) ;
#89986=CARTESIAN_POINT ( 'NONE',  ( 4.620051286339034391, -286.5088600877796807, -332.9519976615662813 ) ) ;
#89987=CARTESIAN_POINT ( 'NONE',  ( 13.49817791269440548, -274.6218043813393024, -217.9749861794490471 ) ) ;
#89988=CARTESIAN_POINT ( 'NONE',  ( 5.557323458068381683, -288.4884333716127003, -334.3038562360549690 ) ) ;
#89989=CARTESIAN_POINT ( 'NONE',  ( -20.98175107099430647, -300.2358698884595469, -195.0004213312810180 ) ) ;
#89990=CARTESIAN_POINT ( 'NONE',  ( -96.23156543239005600, -293.9168872290219383, -316.5348355649385326 ) ) ;
#89991=CARTESIAN_POINT ( 'NONE',  ( -31.65845397940219286, -282.1793319711410390, -347.0024177934992053 ) ) ;
#89994=CARTESIAN_POINT ( 'NONE',  ( -105.6853938518041076, -276.9585912438295736, -239.3474525068313312 ) ) ;
#89996=CARTESIAN_POINT ( 'NONE',  ( -55.09361898898775678, -290.6136367259565532, -199.1431435632293017 ) ) ;
#89999=CARTESIAN_POINT ( 'NONE',  ( -80.66580624260511456, -289.4648332342621870, -209.0763803563716010 ) ) ;
#90000=CARTESIAN_POINT ( 'NONE',  ( -6.253936451024444843, -275.9883323341943537, -203.5460096308692926 ) ) ;
#90001=CARTESIAN_POINT ( 'NONE',  ( 22.07661768964510429, -283.6267616130615465, -318.4241436015711884 ) ) ;
#90002=CARTESIAN_POINT ( 'NONE',  ( 29.00626007061389089, -296.8988656039310285, -195.0281631133275084 ) ) ;
#90003=CARTESIAN_POINT ( 'NONE',  ( -94.28501196460319989, -283.9064458894444556, -316.0587792790577737 ) ) ;
#90004=CARTESIAN_POINT ( 'NONE',  ( -54.36531900083412694, -275.2544331140441045, -198.7680225340782556 ) ) ;
#90005=CARTESIAN_POINT ( 'NONE',  ( 7.421663323858610717, -275.4835860584792044, -212.4919291262028196 ) ) ;
#90006=CARTESIAN_POINT ( 'NONE',  ( 33.72245909192765367, -283.8642270597196102, -294.4994570755767427 ) ) ;
#90009=CARTESIAN_POINT ( 'NONE',  ( 39.23683374338022389, -293.4922253118551794, -278.8969769189378667 ) ) ;
#90010=CARTESIAN_POINT ( 'NONE',  ( -106.1227554609115771, -286.9142439715722048, -241.2279264058203694 ) ) ;
#90012=CARTESIAN_POINT ( 'NONE',  ( -115.3288506153726871, -270.2666405000204009, -252.5284128619063608 ) ) ;
#90013=CARTESIAN_POINT ( 'NONE',  ( -51.29335182039595509, -276.4233504259822780, -345.9224191563960176 ) ) ;
#90015=CARTESIAN_POINT ( 'NONE',  ( -111.7881649066637095, -288.7466284839798050, -286.6142500018415831 ) ) ;
#90016=CARTESIAN_POINT ( 'NONE',  ( -100.2108334420428832, -286.5981973201796791, -231.8167487287633719 ) ) ;
#90018=CARTESIAN_POINT ( 'NONE',  ( -70.89239331583017645, -279.2612618837947593, -336.3332712183571971 ) ) ;
#90019=CARTESIAN_POINT ( 'NONE',  ( -49.27078224464337808, -287.3283742385361279, -194.8339336776473374 ) ) ;
#90020=CARTESIAN_POINT ( 'NONE',  ( -30.09378542254856370, -282.1438988379376269, -195.6604158146076884 ) ) ;
#90021=CARTESIAN_POINT ( 'NONE',  ( 39.55419714377931939, -275.6572572191269614, -265.4376621109302619 ) ) ;
#90022=CARTESIAN_POINT ( 'NONE',  ( -84.86804626794169337, -277.5201096972257346, -331.0114285673242307 ) ) ;
#90023=CARTESIAN_POINT ( 'NONE',  ( -72.36368689922639419, -299.5051649154558504, -204.6596937049019402 ) ) ;
#90025=CARTESIAN_POINT ( 'NONE',  ( -85.33152481854864391, -281.9090924074130839, -210.2361428286349110 ) ) ;
#90027=CARTESIAN_POINT ( 'NONE',  ( -23.61459040309954105, -296.3618478091602242, -194.6006057249171022 ) ) ;
#90029=CARTESIAN_POINT ( 'NONE',  ( -69.28397759739200978, -276.9917183236604501, -336.0840179051645578 ) ) ;
#90030=CARTESIAN_POINT ( 'NONE',  ( -94.79886426350851991, -274.4467380231901075, -219.6986761869628424 ) ) ;
#90031=CARTESIAN_POINT ( 'NONE',  ( 28.09813090857735673, -281.1379961476027916, -310.5922256237240617 ) ) ;
#90032=CARTESIAN_POINT ( 'NONE',  ( 16.69924425416339631, -288.5944773308765434, -219.7701927582697579 ) ) ;
#90033=CARTESIAN_POINT ( 'NONE',  ( -92.18511600274811713, -297.3387870389506702, -323.4168197256554436 ) ) ;
#90034=CARTESIAN_POINT ( 'NONE',  ( -39.08335000664671099, -296.2786235757576492, -346.9442452079462669 ) ) ;
#90035=CARTESIAN_POINT ( 'NONE',  ( -16.95706390093824112, -294.3160089804863446, -198.3037731900492133 ) ) ;
#90036=CARTESIAN_POINT ( 'NONE',  ( -70.53102447828852917, -277.6134202975084690, -203.2760907243010138 ) ) ;
#90037=CARTESIAN_POINT ( 'NONE',  ( 3.473493612593856028, -282.5253630614609506, -208.0462942103282273 ) ) ;
#90038=CARTESIAN_POINT ( 'NONE',  ( -58.28699278625388303, -295.8591700093917893, -198.9285700023416155 ) ) ;
#90039=CARTESIAN_POINT ( 'NONE',  ( -113.5540968977842482, -286.1209057257423751, -272.8437134375274127 ) ) ;
#90040=CARTESIAN_POINT ( 'NONE',  ( 30.25209705113452685, -286.0917412910500275, -241.8517075044405544 ) ) ;
#90041=CARTESIAN_POINT ( 'NONE',  ( -88.13691865063097453, -231.3408449674847702, -347.3187200103926102 ) ) ;
#90043=CARTESIAN_POINT ( 'NONE',  ( 34.58897289824625432, -287.0493038545163813, -257.5033832534419389 ) ) ;
#90045=CARTESIAN_POINT ( 'NONE',  ( -63.79245144485228280, -284.4687785119766090, -342.3461877144193863 ) ) ;
#90046=CARTESIAN_POINT ( 'NONE',  ( 2.938067282751138709, -274.9423024915284941, -209.3939758896729018 ) ) ;
#90047=CARTESIAN_POINT ( 'NONE',  ( 16.03357058837823246, -285.5838686363346142, -215.4148788587463343 ) ) ;
#90048=CARTESIAN_POINT ( 'NONE',  ( -98.09492390808233608, -290.0997878408114161, -223.5366871470241676 ) ) ;
#90049=CARTESIAN_POINT ( 'NONE',  ( 38.94753206673036061, -282.3805555496907118, -261.3655998634806110 ) ) ;
#90050=CARTESIAN_POINT ( 'NONE',  ( -94.45581688582235813, -280.7640520483145679, -219.7579024668104637 ) ) ;
#90051=CARTESIAN_POINT ( 'NONE',  ( 22.50950570810978846, -282.5349472567730231, -318.7924266976679633 ) ) ;
#90052=CARTESIAN_POINT ( 'NONE',  ( -37.30987171927208834, -277.5523547857346784, -200.3611179825600459 ) ) ;
#90053=CARTESIAN_POINT ( 'NONE',  ( 174.8075198983063956, 243.0437970287033522, -179.7850249908958347 ) ) ;
#90055=CARTESIAN_POINT ( 'NONE',  ( 8.728621298072505752, -278.4196222335515358, -329.3979537630773393 ) ) ;
#90056=CARTESIAN_POINT ( 'NONE',  ( -114.3264802394368189, -272.8779462956648558, -270.3652661221577205 ) ) ;
#90057=CARTESIAN_POINT ( 'NONE',  ( 23.92059713507495999, -280.1536162727486499, -313.0082484570966130 ) ) ;
#90058=CARTESIAN_POINT ( 'NONE',  ( 0.06149831950429140298, -296.3215892981411912, -336.5196919456309388 ) ) ;
#90059=CARTESIAN_POINT ( 'NONE',  ( -58.44558161531324458, -294.6808956684941450, -340.3505375693898714 ) ) ;
#90060=CARTESIAN_POINT ( 'NONE',  ( -98.29566159531329106, -290.6870168510663461, -223.3915173916311403 ) ) ;
#90063=CARTESIAN_POINT ( 'NONE',  ( -101.8094543688281135, -295.6686885890848089, -229.3426470773057417 ) ) ;
#90064=CARTESIAN_POINT ( 'NONE',  ( 20.97723512376344246, -286.5823125567796978, -315.6070307612565102 ) ) ;
#90065=CARTESIAN_POINT ( 'NONE',  ( 36.06294326259726546, -295.5605663584228751, -281.7697388787118484 ) ) ;
#90066=CARTESIAN_POINT ( 'NONE',  ( 22.38261756572735806, -288.2716847834572036, -227.4472063587725472 ) ) ;
#90068=CARTESIAN_POINT ( 'NONE',  ( 38.09179241347295175, -294.3148378761175081, -256.1270596544019327 ) ) ;
#90069=CARTESIAN_POINT ( 'NONE',  ( -108.0898192706969496, -285.2850792517341461, -252.1212693096084934 ) ) ;
#90070=CARTESIAN_POINT ( 'NONE',  ( -109.9741202492437537, -295.0389716840304573, -294.7032679612080415 ) ) ;
#90071=CARTESIAN_POINT ( 'NONE',  ( -99.08096175945159700, -291.9645896086000221, -224.5960691673709277 ) ) ;
#90072=CARTESIAN_POINT ( 'NONE',  ( -111.5750778233228715, -291.2985384042939927, -250.0890304602676508 ) ) ;
#90073=CARTESIAN_POINT ( 'NONE',  ( -108.6622656024757703, -290.5127488894129328, -285.9876803642017649 ) ) ;
#90075=DIRECTION ( 'NONE',  ( -1.000000000000000000, -0.000000000000000000, -0.000000000000000000 ) ) ;
#90076=CARTESIAN_POINT ( 'NONE',  ( -20.86902814125024719, -300.1166924632333917, -194.5911552220985072 ) ) ;
#90077=CARTESIAN_POINT ( 'NONE',  ( -66.06402550845980670, -272.4794651163252865, -199.3326804433910979 ) ) ;
#90078=CARTESIAN_POINT ( 'NONE',  ( 34.45899735771880046, -280.8013993939400734, -284.8487499001383298 ) ) ;
#90080=CARTESIAN_POINT ( 'NONE',  ( 35.67354879588813077, -274.7523419694737754, -245.9382336360603460 ) ) ;
#90081=CARTESIAN_POINT ( 'NONE',  ( -109.5680933949462883, -294.8400185573922272, -285.0546890491760337 ) ) ;
#90082=CARTESIAN_POINT ( 'NONE',  ( -21.36446662396460283, -278.7056433737603811, -342.9094662571563390 ) ) ;
#90083=CARTESIAN_POINT ( 'NONE',  ( 24.08755217628629097, -273.1214950897380049, -228.6572265365895475 ) ) ;
#90084=CARTESIAN_POINT ( 'NONE',  ( -109.4385927434285009, -297.9385651161336455, -256.5402513225126881 ) ) ;
#90085=CARTESIAN_POINT ( 'NONE',  ( -88.35065948004125858, -298.3969179446072530, -217.6374811047282094 ) ) ;
#90087=CARTESIAN_POINT ( 'NONE',  ( -100.8938457658708501, -298.7113467824224244, -228.2949275043332023 ) ) ;
#90088=CARTESIAN_POINT ( 'NONE',  ( -98.22295295006043148, -271.1755381684280337, -225.8687767058872282 ) ) ;
#90089=CARTESIAN_POINT ( 'NONE',  ( 30.92061690884715475, -293.8547217613084399, -244.2048808540021128 ) ) ;
#90090=CARTESIAN_POINT ( 'NONE',  ( -4.554374849586840135, -291.0675422885425405, -204.4656237401924272 ) ) ;
#90092=CARTESIAN_POINT ( 'NONE',  ( 39.56917834748387719, -276.0187144069889200, -268.3010997361222962 ) ) ;
#90093=CARTESIAN_POINT ( 'NONE',  ( -100.7188197837267580, -273.2164235174000169, -234.0332193051329739 ) ) ;
#90094=CARTESIAN_POINT ( 'NONE',  ( 36.06928846079339479, -283.3140484478532244, -253.2976408231910739 ) ) ;
#90096=CARTESIAN_POINT ( 'NONE',  ( -33.10292009630843069, -281.6846740888414615, -346.7635073191975721 ) ) ;
#90098=CARTESIAN_POINT ( 'NONE',  ( -105.3678443114821590, -283.3882811167611067, -297.4257394242372925 ) ) ;
#90099=CARTESIAN_POINT ( 'NONE',  ( -63.30328705811949419, -281.3894433031901485, -340.9020594997853664 ) ) ;
#90100=CARTESIAN_POINT ( 'NONE',  ( 12.13051257253169268, -274.9229138450200480, -324.9084561355986125 ) ) ;
#90101=CARTESIAN_POINT ( 'NONE',  ( -56.69646648405463907, -281.8029284398158438, -197.8483490588826044 ) ) ;
#90104=CARTESIAN_POINT ( 'NONE',  ( -89.59924740339535276, -271.7303822857220439, -214.8310865714975364 ) ) ;
#90105=CARTESIAN_POINT ( 'NONE',  ( -93.81612771484273594, -279.8646018512585556, -319.9662332155795070 ) ) ;
#90107=CARTESIAN_POINT ( 'NONE',  ( -112.9009035535466694, -286.4767408517752756, -270.0133064719049685 ) ) ;
#90110=CARTESIAN_POINT ( 'NONE',  ( -38.08263916034813690, -287.0612442873232908, -345.3700619854940896 ) ) ;
#90112=CARTESIAN_POINT ( 'NONE',  ( -92.13113289799510142, -296.0417140836379986, -221.5221114184148519 ) ) ;
#90113=CARTESIAN_POINT ( 'NONE',  ( -103.9642223943870789, -288.2554163740471154, -303.1071865146585651 ) ) ;
#90114=CARTESIAN_POINT ( 'NONE',  ( -104.9628119525177112, -256.0684274861638983, -326.9234398911233939 ) ) ;
#90115=CARTESIAN_POINT ( 'NONE',  ( -104.5719721256332946, -294.1120329261154325, -303.7214697279811162 ) ) ;
#90116=CARTESIAN_POINT ( 'NONE',  ( 2.396614496387613702, -285.0544049508075659, -205.2183969541654278 ) ) ;
#90117=CARTESIAN_POINT ( 'NONE',  ( -6.452979259716959959, -282.0648534210299658, -203.3224978476007152 ) ) ;
#90118=CARTESIAN_POINT ( 'NONE',  ( -70.05446133020546995, -281.7169623758215948, -338.9600048021335965 ) ) ;
#90119=CARTESIAN_POINT ( 'NONE',  ( -0.9914430039996633415, -288.5555535167002290, -333.7253754827576699 ) ) ;
#90120=CARTESIAN_POINT ( 'NONE',  ( -106.0710654899730940, -280.3275246294902558, -243.9190744701859046 ) ) ;
#90121=CARTESIAN_POINT ( 'NONE',  ( 5.008326495467926520, -281.4440702163716423, -210.7031179196456492 ) ) ;
#90123=CARTESIAN_POINT ( 'NONE',  ( 9.231606064393066191, -290.3964007067284570, -329.6671498845664701 ) ) ;
#90124=CARTESIAN_POINT ( 'NONE',  ( -114.1602446862054023, -272.9571022064550334, -264.6320451274926882 ) ) ;
#90126=CARTESIAN_POINT ( 'NONE',  ( -73.94486433745520060, -273.5800940724460020, -202.5581494274476029 ) ) ;
#90127=CARTESIAN_POINT ( 'NONE',  ( 24.69450874071718971, -294.9681996804666824, -228.8477997341847754 ) ) ;
#90129=CARTESIAN_POINT ( 'NONE',  ( 35.78497577281001440, -278.2662352645559167, -287.0191576251351080 ) ) ;
#90130=EDGE_LOOP ( 'NONE', ( #19576, #67716 ) ) ;
#90131=CARTESIAN_POINT ( 'NONE',  ( 37.11183059700131537, -273.4196546579663618, -260.0315396234426544 ) ) ;
#90133=CARTESIAN_POINT ( 'NONE',  ( -65.23003479733981180, -296.0937110755624531, -199.3915327245204310 ) ) ;
#90134=CARTESIAN_POINT ( 'NONE',  ( -32.67625149399010809, -273.4610545259048422, -197.3956698614260574 ) ) ;
#90136=CARTESIAN_POINT ( 'NONE',  ( -105.3503269531424849, -292.4509758920632407, -241.8463026787514423 ) ) ;
#90137=CARTESIAN_POINT ( 'NONE',  ( 12.61696937742673263, -284.1042407086167714, -324.9697743730834532 ) ) ;
#90138=CARTESIAN_POINT ( 'NONE',  ( -111.7476824061083391, -292.1965662743479584, -252.9727282709146152 ) ) ;
#90139=CARTESIAN_POINT ( 'NONE',  ( -97.08901479694810632, -292.5115170597400720, -222.5745438735997936 ) ) ;
#90140=CARTESIAN_POINT ( 'NONE',  ( 3.814636806671683367, -294.3140373766194671, -330.6533723325371170 ) ) ;
#90141=CARTESIAN_POINT ( 'NONE',  ( 31.79581338937473944, -289.1710774746628658, -241.1577655107864473 ) ) ;
#90142=CARTESIAN_POINT ( 'NONE',  ( -4.161912957332621232, -282.7934014040489501, -339.8601504212729196 ) ) ;
#90143=CARTESIAN_POINT ( 'NONE',  ( -110.2264170385144837, -294.8885843840683378, -250.2398400608089730 ) ) ;
#90144=CARTESIAN_POINT ( 'NONE',  ( 0.8665143576031041350, -282.3904208385632728, -337.2279194807567251 ) ) ;
#90145=CARTESIAN_POINT ( 'NONE',  ( 4.067037680883670347, -278.4710852926170332, -332.4671823712152445 ) ) ;
#90147=CARTESIAN_POINT ( 'NONE',  ( -6.941161984400275209, -285.1233781216987495, -333.4151289067050357 ) ) ;
#90149=CARTESIAN_POINT ( 'NONE',  ( -106.4591617536603252, -276.2874856991006709, -301.5224302475011200 ) ) ;
#90151=CARTESIAN_POINT ( 'NONE',  ( -37.54698722155948332, -282.5624774651789153, -343.4348082593910476 ) ) ;
#90152=CARTESIAN_POINT ( 'NONE',  ( -99.11680002086713159, -280.3621460004630421, -225.0416702303547822 ) ) ;
#90153=CARTESIAN_POINT ( 'NONE',  ( 39.11202683624916432, -286.6974951852448044, -277.2638598844710032 ) ) ;
#90154=CARTESIAN_POINT ( 'NONE',  ( -55.27934195559270592, -293.5783764819179282, -198.5543284943716174 ) ) ;
#90155=CARTESIAN_POINT ( 'NONE',  ( 6.755258838090697715, -276.2406654620227755, -208.1521992418941807 ) ) ;
#90156=CARTESIAN_POINT ( 'NONE',  ( 31.41946182506521268, -277.3021462103484396, -304.0258547448161153 ) ) ;
#90157=CARTESIAN_POINT ( 'NONE',  ( -94.45436295300844165, -277.7431814912611685, -315.8469381730821510 ) ) ;
#90158=CARTESIAN_POINT ( 'NONE',  ( 98.54881674486404108, -301.7573013711235035, -195.4813331363455120 ) ) ;
#90159=CARTESIAN_POINT ( 'NONE',  ( -35.87256191074403233, -284.0704663282263596, -195.5422028401620196 ) ) ;
#90160=CARTESIAN_POINT ( 'NONE',  ( 29.45939891080023898, -292.7217262870388481, -232.1072625082411491 ) ) ;
#90161=CARTESIAN_POINT ( 'NONE',  ( -109.1051765401954583, -291.8237004611193015, -296.1385909104058669 ) ) ;
#90162=CARTESIAN_POINT ( 'NONE',  ( -44.31598193566112087, -290.8823355036425369, -197.3334762996184963 ) ) ;
#90164=CARTESIAN_POINT ( 'NONE',  ( -16.76768863807515331, -290.8875847654112476, -196.7722849802970302 ) ) ;
#90165=CARTESIAN_POINT ( 'NONE',  ( -17.42275272762526583, -291.9829429016224935, -200.0566551615702906 ) ) ;
#90167=CARTESIAN_POINT ( 'NONE',  ( -75.49790889335865529, -290.6284404359536779, -336.8862729430172749 ) ) ;
#90168=CARTESIAN_POINT ( 'NONE',  ( -110.4939043938701104, -279.1998073312115025, -270.6467192223136067 ) ) ;
#90169=CARTESIAN_POINT ( 'NONE',  ( -93.42726370851575268, -296.1891288855873086, -217.9778211481304879 ) ) ;
#90170=CARTESIAN_POINT ( 'NONE',  ( -67.15720418183705931, -286.3227829624628384, -199.4784790307031130 ) ) ;
#90171=CARTESIAN_POINT ( 'NONE',  ( 39.58341944732033113, -287.9361783288266565, -274.4175880791987652 ) ) ;
#90172=CARTESIAN_POINT ( 'NONE',  ( -108.3870707587850291, -285.1085875285713769, -253.4358932869931778 ) ) ;
#90173=CARTESIAN_POINT ( 'NONE',  ( -31.41437309758456919, -124.1952521004627670, -364.2598719284257527 ) ) ;
#90174=CARTESIAN_POINT ( 'NONE',  ( 187.7861472146279311, 270.9134355758718584, -138.7283278565937508 ) ) ;
#90175=CARTESIAN_POINT ( 'NONE',  ( 83.88734089079683542, 81.93120406021242275, -298.7933839319709364 ) ) ;
#90176=CARTESIAN_POINT ( 'NONE',  ( -56.65261662564040535, -276.5045677411774818, -340.9806545945097582 ) ) ;
#90177=CARTESIAN_POINT ( 'NONE',  ( 35.14937760062440475, -274.3279059302714131, -259.3554836774226260 ) ) ;
#90178=CARTESIAN_POINT ( 'NONE',  ( -99.86787969626108463, -296.6543971366326105, -225.5280523731308335 ) ) ;
#90179=CARTESIAN_POINT ( 'NONE',  ( 203.7387371057621976, 292.1034155335181595, -68.30586525936504927 ) ) ;
#90180=CARTESIAN_POINT ( 'NONE',  ( -39.96293960670030287, -275.7692390514889667, -346.8360344649427702 ) ) ;
#90181=CARTESIAN_POINT ( 'NONE',  ( -100.1521190306095974, -274.8452414421937533, -231.2098052351783508 ) ) ;
#90183=CARTESIAN_POINT ( 'NONE',  ( -109.4788638772821940, -290.8907649120752694, -282.0250181196129233 ) ) ;
#90184=CARTESIAN_POINT ( 'NONE',  ( -87.36490513066451058, -298.1782784623947009, -211.9656929289267850 ) ) ;
#90185=CARTESIAN_POINT ( 'NONE',  ( -113.7144538629193846, -297.1610611753389435, -261.0482564390395623 ) ) ;
#90186=CARTESIAN_POINT ( 'NONE',  ( 21.32773324413360072, -294.3278788925558160, -313.7995524882792324 ) ) ;
#90188=CARTESIAN_POINT ( 'NONE',  ( -95.92217566525884820, -279.8194266966205532, -318.1060205293470062 ) ) ;
#90189=CARTESIAN_POINT ( 'NONE',  ( 33.50680871513438319, -281.4434666549176995, -300.4974095092120479 ) ) ;
#90190=CARTESIAN_POINT ( 'NONE',  ( -24.27588793701781000, -277.8226245302699908, -342.4730785326017894 ) ) ;
#90191=CARTESIAN_POINT ( 'NONE',  ( 20.06954850271101165, -277.9940718067817897, -320.1595542729565977 ) ) ;
#90192=CARTESIAN_POINT ( 'NONE',  ( -106.9550501378554799, -271.3505882487010581, -246.1807695084043530 ) ) ;
#90194=CARTESIAN_POINT ( 'NONE',  ( -72.84014796095637223, -277.7030459553524224, -334.1631175055009066 ) ) ;
#90195=CARTESIAN_POINT ( 'NONE',  ( -32.70258911654635625, -274.9120186768099074, -193.6496411329764555 ) ) ;
#90196=CARTESIAN_POINT ( 'NONE',  ( -15.11164831457424107, -287.4550957492417638, -343.6225398705749967 ) ) ;
#90197=CARTESIAN_POINT ( 'NONE',  ( -77.78506792377260126, -275.5091014192090597, -207.1999380638553703 ) ) ;
#90199=CARTESIAN_POINT ( 'NONE',  ( -15.81387265384110918, -287.9637265144304479, -340.3365456402897280 ) ) ;
#90200=CARTESIAN_POINT ( 'NONE',  ( -109.2106551898552027, -283.5523808708134652, -297.8621645647637592 ) ) ;
#90201=CARTESIAN_POINT ( 'NONE',  ( 27.73553469996999610, -280.2664762417829820, -305.6162951674692749 ) ) ;
#90202=CARTESIAN_POINT ( 'NONE',  ( 24.18507444310836974, -279.5705762980783220, -229.8980252222388856 ) ) ;
#90203=CARTESIAN_POINT ( 'NONE',  ( -52.35594776973218245, -283.9382260207681838, -197.4509913697332593 ) ) ;
#90204=CARTESIAN_POINT ( 'NONE',  ( -79.64505473336781449, -291.6235539402017594, -332.3540981352957715 ) ) ;
#90205=CARTESIAN_POINT ( 'NONE',  ( -89.76789227409565797, -280.4973907152653965, -218.9215265224820541 ) ) ;
#90207=CARTESIAN_POINT ( 'NONE',  ( 38.47990406833412891, -280.0543012940727863, -278.4540283201876605 ) ) ;
#90208=CARTESIAN_POINT ( 'NONE',  ( -33.66360306652134682, -294.0986121181003341, -195.4513572526384735 ) ) ;
#90209=CARTESIAN_POINT ( 'NONE',  ( -98.59751601564781254, -277.3974082529711609, -225.3758587141356031 ) ) ;
#90210=CARTESIAN_POINT ( 'NONE',  ( -41.85460081388423248, -277.7618990135222248, -343.3362319250621226 ) ) ;
#90211=CARTESIAN_POINT ( 'NONE',  ( -107.5804948036154656, -286.2035275333274171, -297.2742918177161187 ) ) ;
#90212=DIRECTION ( 'NONE',  ( 0.9951408606192336803, 0.000000000000000000, -0.09846150276128748380 ) ) ;
#90213=CARTESIAN_POINT ( 'NONE',  ( -112.9489458325655136, -292.4611462319977591, -271.2369360244861696 ) ) ;
#90214=CARTESIAN_POINT ( 'NONE',  ( 38.92898483075529725, -286.8715371414518813, -280.1128547203847461 ) ) ;
#90215=CARTESIAN_POINT ( 'NONE',  ( -41.61905078916150558, -290.3973912909737010, -196.6347808735201852 ) ) ;
#90217=CARTESIAN_POINT ( 'NONE',  ( 32.53589558288029338, -273.9349542496498771, -247.4296587769936195 ) ) ;
#90218=CARTESIAN_POINT ( 'NONE',  ( 23.93947580448152124, -292.2661274993499774, -312.3494546677990797 ) ) ;
#90220=CARTESIAN_POINT ( 'NONE',  ( 37.64750106673213281, -291.8538617524871484, -256.2427803231421990 ) ) ;
#90221=CARTESIAN_POINT ( 'NONE',  ( -102.9588975220734852, -286.6064475842487695, -236.5850344434279862 ) ) ;
#90222=CARTESIAN_POINT ( 'NONE',  ( -20.73992347687352833, -287.0818639099150005, -344.5659556676834541 ) ) ;
#90223=CARTESIAN_POINT ( 'NONE',  ( 33.22992185544049448, -288.7031185475520942, -249.4595447327372995 ) ) ;
#90225=CARTESIAN_POINT ( 'NONE',  ( 32.82193134830651360, -288.0807793293030272, -249.5885461554855738 ) ) ;
#90226=EDGE_CURVE ( 'NONE', #47196, #64985, #62903, .T. ) ;
#90227=CARTESIAN_POINT ( 'NONE',  ( 38.01029806876059780, -295.4951506261967893, -267.4739222729283483 ) ) ;
#90228=CARTESIAN_POINT ( 'NONE',  ( -112.6462317283272938, -276.5451384234661987, -277.1764000091938556 ) ) ;
#90229=CARTESIAN_POINT ( 'NONE',  ( -74.08302051657516074, -277.8599109470321196, -338.0209206272429583 ) ) ;
#90230=CARTESIAN_POINT ( 'NONE',  ( 22.84335777169875925, -291.0114167651252615, -224.6553238796714140 ) ) ;
#90231=CARTESIAN_POINT ( 'NONE',  ( -86.80472195717005945, -279.3863449120256064, -211.2796780886763770 ) ) ;
#90232=CARTESIAN_POINT ( 'NONE',  ( -37.85865255701175869, -300.0255354181899179, -195.7181037938501333 ) ) ;
#90234=CARTESIAN_POINT ( 'NONE',  ( -110.6810105371885982, -282.3496828225431159, -286.1176294838675176 ) ) ;
#90236=CARTESIAN_POINT ( 'NONE',  ( -111.1924004894778051, -276.7959876254700475, -262.3241402486000879 ) ) ;
#90237=CARTESIAN_POINT ( 'NONE',  ( 36.03345623882090365, -279.3518397112863454, -254.7726022256022134 ) ) ;
#90239=CARTESIAN_POINT ( 'NONE',  ( -73.78293023564260977, -276.0068072159758117, -337.4188423444060163 ) ) ;
#90240=CARTESIAN_POINT ( 'NONE',  ( -70.01421983127275439, -297.0107569983521785, -336.4157484848395825 ) ) ;
#90241=CARTESIAN_POINT ( 'NONE',  ( -21.80210880432005993, -281.7778021113119280, -345.4611420196619065 ) ) ;
#90242=CARTESIAN_POINT ( 'NONE',  ( -107.8260178613610947, -297.2314009983613801, -290.2450160460394954 ) ) ;
#90243=CARTESIAN_POINT ( 'NONE',  ( -62.69749977286563336, -299.0440613989799203, -198.1781442523023031 ) ) ;
#90244=CARTESIAN_POINT ( 'NONE',  ( -16.63060276863775755, -273.9938007425339492, -200.2859830649728679 ) ) ;
#90245=CARTESIAN_POINT ( 'NONE',  ( -0.2902045951222534947, -294.5449658596472204, -205.1374507274707639 ) ) ;
#90246=CARTESIAN_POINT ( 'NONE',  ( 38.28978479963161874, -287.5380813172204739, -255.9084887355259070 ) ) ;
#90247=CARTESIAN_POINT ( 'NONE',  ( 5.158502412749834676, -274.6235960332911077, -333.0830301226208690 ) ) ;
#90248=CARTESIAN_POINT ( 'NONE',  ( -62.76565589592060235, -289.2073230599058888, -343.0991544958789632 ) ) ;
#90250=CARTESIAN_POINT ( 'NONE',  ( 25.89318396655322729, -287.1175450148280675, -307.4039760413180602 ) ) ;
#90251=CARTESIAN_POINT ( 'NONE',  ( -101.4916234322722772, -289.0738365933872842, -231.4050520080278943 ) ) ;
#90253=CARTESIAN_POINT ( 'NONE',  ( 68.56402772857219929, 46.98157435473511612, -321.4867780223927980 ) ) ;
#90254=CARTESIAN_POINT ( 'NONE',  ( -66.35923439008259095, -288.9501479939425508, -337.4671855449669238 ) ) ;
#90256=CARTESIAN_POINT ( 'NONE',  ( -97.40381903799490715, -286.1353716648494583, -222.5556571405401485 ) ) ;
#90257=CARTESIAN_POINT ( 'NONE',  ( -39.19396321485209711, -291.0882250066502479, -193.6057655870010592 ) ) ;
#90258=CARTESIAN_POINT ( 'NONE',  ( 14.60095078737550978, -282.3684854302027816, -214.5359661306991370 ) ) ;
#90259=CARTESIAN_POINT ( 'NONE',  ( -48.06632584490038340, -281.2337519709469120, -194.5561768831846621 ) ) ;
#90260=CARTESIAN_POINT ( 'NONE',  ( -38.88720806377160244, -282.9053596033864437, -343.3572467925595220 ) ) ;
#90261=CARTESIAN_POINT ( 'NONE',  ( -68.85521594082125318, -279.4665886444153671, -338.4332954252337231 ) ) ;
#90262=CARTESIAN_POINT ( 'NONE',  ( -113.1391160217790457, -296.7216824773335020, -256.8056119485592603 ) ) ;
#90263=CARTESIAN_POINT ( 'NONE',  ( -94.17031542830721946, -274.5232084580507603, -223.7393757060845871 ) ) ;
#90264=CARTESIAN_POINT ( 'NONE',  ( -14.31559698186996421, -290.3723170832461733, -199.3565732352207647 ) ) ;
#90265=CARTESIAN_POINT ( 'NONE',  ( -104.7382635720461934, -271.7370843226956936, -241.1663573600054065 ) ) ;
#90267=CARTESIAN_POINT ( 'NONE',  ( -95.39291326371389346, -285.8262890322477574, -316.9793568464417604 ) ) ;
#90268=CARTESIAN_POINT ( 'NONE',  ( 22.05599015673160679, -295.2857992579992015, -318.8936639282692340 ) ) ;
#90269=CARTESIAN_POINT ( 'NONE',  ( -81.54679794574521168, -286.0836324178754921, -212.1391118786113168 ) ) ;
#90270=CARTESIAN_POINT ( 'NONE',  ( 3.366532553764151281, -275.5783129631894894, -335.5056328408796276 ) ) ;
#90271=CARTESIAN_POINT ( 'NONE',  ( -84.21079868002868807, -292.0783456313117199, -209.3300742823917631 ) ) ;
#90272=CARTESIAN_POINT ( 'NONE',  ( -102.9586576800951008, -283.1933971071168799, -232.3791388229669792 ) ) ;
#90273=CARTESIAN_POINT ( 'NONE',  ( -34.96531909373578628, -292.4144799636879952, -193.4058042189810749 ) ) ;
#90274=CARTESIAN_POINT ( 'NONE',  ( -39.95452290089063041, -289.4190355840145230, -343.3850933968739696 ) ) ;
#90277=CARTESIAN_POINT ( 'NONE',  ( -110.8433564205054438, -271.0408464140099909, -283.6640628832823268 ) ) ;
#90278=CARTESIAN_POINT ( 'NONE',  ( -78.16799930467063007, -287.0338436876424453, -205.8946844890710111 ) ) ;
#90279=CARTESIAN_POINT ( 'NONE',  ( 40.65961533371913106, -272.8380690714490129, -252.5904736702033802 ) ) ;
#90281=CARTESIAN_POINT ( 'NONE',  ( 21.58561121256696680, -279.8633862053048915, -226.7303755778752645 ) ) ;
#90282=CARTESIAN_POINT ( 'NONE',  ( -1.481342910053283335, -276.2565674700657041, -338.4770417580498361 ) ) ;
#90283=CARTESIAN_POINT ( 'NONE',  ( -97.90403835941212662, -281.1523823480698638, -226.4039613800688642 ) ) ;
#90284=CARTESIAN_POINT ( 'NONE',  ( -10.82389337143313135, -93.05637620313754610, -358.2402470118966562 ) ) ;
#90285=CARTESIAN_POINT ( 'NONE',  ( -78.85494278081915809, -282.1747055079428605, -334.5113866990816973 ) ) ;
#90286=CARTESIAN_POINT ( 'NONE',  ( -60.46473692186032878, -283.7708841519874454, -199.3880810574634950 ) ) ;
#90287=CARTESIAN_POINT ( 'NONE',  ( -33.42247641351010401, -299.8607127602575133, -194.3732890516851910 ) ) ;
#90288=CARTESIAN_POINT ( 'NONE',  ( -77.97876766186865893, -296.1066482066365779, -331.1397416483043799 ) ) ;
#90290=CARTESIAN_POINT ( 'NONE',  ( 27.93216489230453448, -291.7807978776816640, -236.5888509290503237 ) ) ;
#90291=CARTESIAN_POINT ( 'NONE',  ( 23.44257852655138308, -276.8335429644004080, -317.4843262545308562 ) ) ;
#90292=CARTESIAN_POINT ( 'NONE',  ( 34.12134524492419985, -275.3547811567860890, -255.3993167324521494 ) ) ;
#90293=CARTESIAN_POINT ( 'NONE',  ( 17.87662385336003013, -273.7401728499644378, -217.0642995870800291 ) ) ;
#90295=CARTESIAN_POINT ( 'NONE',  ( 9.741099533415315648, -272.6996006410201971, -211.9152923815999543 ) ) ;
#90296=CARTESIAN_POINT ( 'NONE',  ( -0.9705319950128667994, -296.0043371559549996, -337.5751797897855795 ) ) ;
#90299=CARTESIAN_POINT ( 'NONE',  ( -1.087228655259989685, -283.6384841326533319, -334.0779868018282741 ) ) ;
#90300=CARTESIAN_POINT ( 'NONE',  ( 36.68514615086283470, -283.0943330725252167, -253.1575948953936859 ) ) ;
#90301=CARTESIAN_POINT ( 'NONE',  ( -101.0761317332694205, -284.3911811793102515, -234.4549573645665816 ) ) ;
#90302=CARTESIAN_POINT ( 'NONE',  ( -59.45389679821642659, -275.7431620975099804, -340.7705716957821096 ) ) ;
#90303=CARTESIAN_POINT ( 'NONE',  ( -34.78059007177041906, -284.8800885926299316, -344.5647762741884321 ) ) ;
#90304=CARTESIAN_POINT ( 'NONE',  ( -110.1802725726846148, -276.8857796841296590, -281.5526378572948261 ) ) ;
#90306=CARTESIAN_POINT ( 'NONE',  ( -114.2231699715874953, -279.3392566174510989, -271.6159845739180696 ) ) ;
#90309=CARTESIAN_POINT ( 'NONE',  ( -93.02823615882769559, -287.1240718687753315, -218.9099358403580027 ) ) ;
#90311=CARTESIAN_POINT ( 'NONE',  ( -39.70447306423596956, -294.2797126374510981, -343.4968896658414224 ) ) ;
#90312=CARTESIAN_POINT ( 'NONE',  ( -101.5942191312459641, -290.4579537820420683, -228.0171874096032809 ) ) ;
#90313=CARTESIAN_POINT ( 'NONE',  ( 34.05350582185366193, -286.0484844918586305, -290.0625849946681001 ) ) ;
#90314=CARTESIAN_POINT ( 'NONE',  ( -16.99165617770425385, -284.8946983804767683, -199.5883189499267303 ) ) ;
#90315=CARTESIAN_POINT ( 'NONE',  ( -108.3614058151910484, -289.0644404839585491, -249.4792877253562153 ) ) ;
#90316=CARTESIAN_POINT ( 'NONE',  ( -66.70440491860692589, -284.6506744658333901, -337.6425996158478711 ) ) ;
#90317=CARTESIAN_POINT ( 'NONE',  ( 15.52685055953734938, -274.3048549042079571, -323.6305749097360831 ) ) ;
#90318=CARTESIAN_POINT ( 'NONE',  ( -3.822688026705792996, -284.8868179811015580, -201.9149022078535154 ) ) ;
#90319=CARTESIAN_POINT ( 'NONE',  ( -3.157811986379429392, -288.5037884096350922, -203.5900097945627465 ) ) ;
#90320=CARTESIAN_POINT ( 'NONE',  ( 36.23435358872315959, -285.3541356054674907, -254.9171253671933073 ) ) ;
#90321=CARTESIAN_POINT ( 'NONE',  ( 28.36746431961739034, -282.9315629165246833, -302.8137459536339975 ) ) ;
#90322=CARTESIAN_POINT ( 'NONE',  ( -41.62988728091504242, -291.1061843201651413, -345.4182782326228107 ) ) ;
#90325=CARTESIAN_POINT ( 'NONE',  ( -78.66854085205032732, -297.5243033608015253, -333.6177890311099645 ) ) ;
#90326=CARTESIAN_POINT ( 'NONE',  ( -68.10394727419324568, -277.6480984868964583, -201.9462293040242002 ) ) ;
#90327=CARTESIAN_POINT ( 'NONE',  ( 13.18000835964080686, -291.9348286519712019, -212.4671131848947994 ) ) ;
#90328=CARTESIAN_POINT ( 'NONE',  ( -90.60933017775367659, -295.6818859337348613, -219.2096358531310614 ) ) ;
#90329=CARTESIAN_POINT ( 'NONE',  ( 20.55921766436886955, -280.8707185380458782, -315.6239857483237188 ) ) ;
#90330=CARTESIAN_POINT ( 'NONE',  ( -31.19693970416748741, -272.2101873814651185, -196.1622624428697179 ) ) ;
#90331=CARTESIAN_POINT ( 'NONE',  ( 20.08956524221319739, -295.5109225487952926, -316.2384998094022421 ) ) ;
#90333=CARTESIAN_POINT ( 'NONE',  ( -111.2436806109478482, -271.3741745718391485, -250.7396404103864995 ) ) ;
#90334=CARTESIAN_POINT ( 'NONE',  ( -4.955047983882035822, -292.8714688989705905, -339.1146034758447172 ) ) ;
#90335=CARTESIAN_POINT ( 'NONE',  ( -49.80624549954305991, -293.3154643216282693, -197.7834499110632009 ) ) ;
#90337=CARTESIAN_POINT ( 'NONE',  ( 21.46233837268349021, -294.9639285873884091, -313.8891179752441758 ) ) ;
#90339=CARTESIAN_POINT ( 'NONE',  ( -96.76331142473912905, -281.9396113719575396, -316.7020169601669863 ) ) ;
#90340=CARTESIAN_POINT ( 'NONE',  ( -55.80330993922925131, -295.2963975017402163, -341.0404718313893113 ) ) ;
#90341=CARTESIAN_POINT ( 'NONE',  ( 34.58750622549786868, -281.9000618070899691, -297.8418252759362304 ) ) ;
#90342=CARTESIAN_POINT ( 'NONE',  ( -67.87686953301690096, -283.1088642971622562, -341.0247417291120087 ) ) ;
#90343=CARTESIAN_POINT ( 'NONE',  ( -108.7080324253075787, -288.2588691537977184, -293.0465819194508299 ) ) ;
#90345=CARTESIAN_POINT ( 'NONE',  ( 36.66361052477951432, -279.7972148318758627, -251.7621462369345409 ) ) ;
#90346=CARTESIAN_POINT ( 'NONE',  ( 27.17727345250740711, -287.0196806989632705, -311.9173560281780055 ) ) ;
#90347=CARTESIAN_POINT ( 'NONE',  ( -36.97128956651225451, -296.6475354380180534, -344.1727519500162202 ) ) ;
#90348=CARTESIAN_POINT ( 'NONE',  ( -25.84060616489625062, -278.3336692868807063, -345.9013796268242800 ) ) ;
#90349=CARTESIAN_POINT ( 'NONE',  ( -30.25611005660749697, -279.8108334134322490, -197.6341914982838830 ) ) ;
#90350=CARTESIAN_POINT ( 'NONE',  ( -5.888878814159318686, -292.6209827031057671, -200.0636878991154788 ) ) ;
#90351=CARTESIAN_POINT ( 'NONE',  ( -90.86538316923216030, -283.3796230072475169, -217.0269867841931841 ) ) ;
#90352=CARTESIAN_POINT ( 'NONE',  ( -66.89641061907894937, -279.4396156094911703, -339.2923862049638046 ) ) ;
#90353=CARTESIAN_POINT ( 'NONE',  ( 35.87667263266076390, -292.6523132273595138, -273.5110069074565331 ) ) ;
#90354=CARTESIAN_POINT ( 'NONE',  ( -102.1094738061161422, -295.0584019353717053, -232.4416868310134703 ) ) ;
#90357=CARTESIAN_POINT ( 'NONE',  ( -12.99364014805401624, -294.2348347125465011, -339.2995436961770110 ) ) ;
#90359=CARTESIAN_POINT ( 'NONE',  ( -82.08285599513421005, -282.9094976428776249, -214.2051214447836571 ) ) ;
#90360=CARTESIAN_POINT ( 'NONE',  ( -109.0122795034231871, -272.1026371911677870, -242.5111566755481647 ) ) ;
#90361=CARTESIAN_POINT ( 'NONE',  ( 35.79890992453862708, -279.4395897272321463, -250.5442946994076863 ) ) ;
#90362=CARTESIAN_POINT ( 'NONE',  ( 21.69885967798633430, -288.2093361042900028, -221.7040468376499405 ) ) ;
#90363=CARTESIAN_POINT ( 'NONE',  ( -75.87054129358756427, -289.4157248156358833, -332.3653791501772048 ) ) ;
#90364=CARTESIAN_POINT ( 'NONE',  ( -69.53700670080370116, -279.0038616006360712, -336.6636209178132049 ) ) ;
#90365=CARTESIAN_POINT ( 'NONE',  ( -73.35934398949902402, -299.3275775620223271, -205.7027593182978364 ) ) ;
#90367=CARTESIAN_POINT ( 'NONE',  ( -45.96992635546732942, -275.9587742842610965, -343.3001819554278882 ) ) ;
#90369=CARTESIAN_POINT ( 'NONE',  ( -29.05819509579903936, -297.8199280375310423, -193.3827149222969126 ) ) ;
#90370=CARTESIAN_POINT ( 'NONE',  ( -111.7444087704486861, -292.4251952944334221, -274.0033251148691420 ) ) ;
#90371=CARTESIAN_POINT ( 'NONE',  ( 0.1646776635978103864, -296.1616022925646234, -336.7064670191150526 ) ) ;
#90374=CARTESIAN_POINT ( 'NONE',  ( -91.75457245208659174, -291.9014077840197388, -221.5250595760859653 ) ) ;
#90376=CARTESIAN_POINT ( 'NONE',  ( -30.78024186626734249, -290.2737031250564996, -194.8290579847819401 ) ) ;
#90377=CARTESIAN_POINT ( 'NONE',  ( -34.05234342206758669, -298.4255600716530807, -193.3820815229926495 ) ) ;
#90378=CARTESIAN_POINT ( 'NONE',  ( -107.6243128501388071, -295.9570737400011353, -290.1712627519395369 ) ) ;
#90381=CARTESIAN_POINT ( 'NONE',  ( -80.13562550161836384, -291.1397549930306923, -333.6023700536939032 ) ) ;
#90382=CARTESIAN_POINT ( 'NONE',  ( 40.64545035920995986, -289.8376638359844719, -252.5284128619064461 ) ) ;
#90383=CARTESIAN_POINT ( 'NONE',  ( -102.6023083257882860, -287.0423280101258570, -233.6340795789281231 ) ) ;
#90384=CARTESIAN_POINT ( 'NONE',  ( -24.25130737657040569, -272.2193692844222710, -196.6287218267999890 ) ) ;
#90385=CARTESIAN_POINT ( 'NONE',  ( -79.69405811200000755, -275.3953687301681725, -209.0809121852981320 ) ) ;
#90386=CARTESIAN_POINT ( 'NONE',  ( -1.729442012136990448, -290.6076750210952468, -204.9778309715839271 ) ) ;
#90387=CARTESIAN_POINT ( 'NONE',  ( -81.80199211890199251, -279.5110740460269767, -331.7092060873821424 ) ) ;
#90388=CARTESIAN_POINT ( 'NONE',  ( 26.94074944044356101, -281.3750257754271047, -305.1700154851422440 ) ) ;
#90389=CARTESIAN_POINT ( 'NONE',  ( -106.0622624743833171, -279.1911556051008461, -304.5243044831680663 ) ) ;
#90390=CARTESIAN_POINT ( 'NONE',  ( -31.09077634398100543, -278.9242592134537517, -193.9612389027497557 ) ) ;
#90391=CARTESIAN_POINT ( 'NONE',  ( 119.9890085633751937, 148.7358962376707439, -260.8480417884134113 ) ) ;
#90392=CARTESIAN_POINT ( 'NONE',  ( 39.08184792331802271, -276.3959431867834269, -262.5922020079913750 ) ) ;
#90393=CARTESIAN_POINT ( 'NONE',  ( -78.48416444828940541, -275.0291402594331203, -206.0960000615810372 ) ) ;
#90394=CARTESIAN_POINT ( 'NONE',  ( -37.30987171927208124, -297.5519495502701943, -345.3611179825600175 ) ) ;
#90398=CARTESIAN_POINT ( 'NONE',  ( -29.12488192841018986, -290.0252483340416916, -343.2082865755819512 ) ) ;
#90399=CARTESIAN_POINT ( 'NONE',  ( 38.59288139358631042, -289.3628087000748792, -274.3471321351187271 ) ) ;
#90400=CARTESIAN_POINT ( 'NONE',  ( -63.86560607265932532, -288.7558257394470047, -338.5356800184054009 ) ) ;
#90401=CARTESIAN_POINT ( 'NONE',  ( -33.72394485042956802, -285.6041901037870616, -193.5077592394279691 ) ) ;
#90403=CARTESIAN_POINT ( 'NONE',  ( 34.54422362365561838, -279.7341205553152577, -253.6621843615318710 ) ) ;
#90404=CARTESIAN_POINT ( 'NONE',  ( 4.327205072108847972, -290.3445182259978310, -331.8606263311714315 ) ) ;
#90405=CARTESIAN_POINT ( 'NONE',  ( 3.761029688458136011, -280.9680863860985482, -331.5887828602889726 ) ) ;
#90406=CARTESIAN_POINT ( 'NONE',  ( -105.9808377428451536, -280.2174440780810301, -243.9523122969912947 ) ) ;
#90407=CARTESIAN_POINT ( 'NONE',  ( -71.67756389271399087, -278.0110926378047225, -334.8658244490279685 ) ) ;
#90408=CARTESIAN_POINT ( 'NONE',  ( -90.49928961750495660, -290.1146560998924997, -215.1306523232821348 ) ) ;
#90409=CARTESIAN_POINT ( 'NONE',  ( -111.3332120467901376, -285.0947679566928628, -291.0834485645143559 ) ) ;
#90410=CARTESIAN_POINT ( 'NONE',  ( -46.50439295085475067, -286.4311645642620761, -193.9702025320064820 ) ) ;
#90411=CARTESIAN_POINT ( 'NONE',  ( -66.55762340021280465, -283.6124466284776986, -337.2733422451516958 ) ) ;
#90413=CARTESIAN_POINT ( 'NONE',  ( 82.64890176555634582, -299.5541904835138780, -197.7570935515976203 ) ) ;
#90414=CARTESIAN_POINT ( 'NONE',  ( -110.3453433170029712, -292.1544968999503453, -290.6286674967419117 ) ) ;
#90415=CARTESIAN_POINT ( 'NONE',  ( 29.13780701110361449, -292.7331104276376550, -308.3332980187386738 ) ) ;
#90416=CARTESIAN_POINT ( 'NONE',  ( 35.82272852617663261, -274.5553545514828784, -266.1373098899807701 ) ) ;
#90417=CARTESIAN_POINT ( 'NONE',  ( -77.03672865549508231, -294.9175268721442080, -336.2836616551266502 ) ) ;
#90418=CARTESIAN_POINT ( 'NONE',  ( -108.7758209300875905, -289.2693709503874402, -252.2025557979152950 ) ) ;
#90419=CARTESIAN_POINT ( 'NONE',  ( -3.898560151428867027, -292.8446945248484781, -336.4020487897673206 ) ) ;
#90420=CARTESIAN_POINT ( 'NONE',  ( -110.3694930110057442, -291.8537121254119029, -263.0077533798935292 ) ) ;
#90422=CARTESIAN_POINT ( 'NONE',  ( 26.50882205886980003, -291.0193906701816786, -230.5998967255951300 ) ) ;
#90423=CARTESIAN_POINT ( 'NONE',  ( -85.29585550121535675, -297.7143839599389139, -328.0941810272661883 ) ) ;
#90424=CARTESIAN_POINT ( 'NONE',  ( 33.25289301502674277, -288.2367111987811086, -250.8723553861403275 ) ) ;
#90426=CARTESIAN_POINT ( 'NONE',  ( 36.30370095453862689, -277.7367860560564168, -286.3827532494691468 ) ) ;
#90427=CARTESIAN_POINT ( 'NONE',  ( -96.75620157317635517, -276.6947032797544352, -318.7337652591716619 ) ) ;
#90428=CARTESIAN_POINT ( 'NONE',  ( -14.85853804091576791, -297.5240962728179284, -193.5255645770875788 ) ) ;
#90429=CARTESIAN_POINT ( 'NONE',  ( 31.20820741809435006, -274.1623476043325809, -298.4058836241657104 ) ) ;
#90430=CARTESIAN_POINT ( 'NONE',  ( -52.08918302576198300, -277.9418988163803874, -197.3438173247801046 ) ) ;
#90431=CARTESIAN_POINT ( 'NONE',  ( 11.80105736291380225, -275.9576610621847976, -215.7755448104324785 ) ) ;
#90432=CARTESIAN_POINT ( 'NONE',  ( -14.84552422774434000, -275.1654575875252249, -343.2199471010634966 ) ) ;
#90434=CARTESIAN_POINT ( 'NONE',  ( -52.67889550529869780, -298.6535656316958693, -198.7733060897125767 ) ) ;
#90436=CARTESIAN_POINT ( 'NONE',  ( -5.061026023153183395, -286.6494641961273828, -338.4661430223707157 ) ) ;
#90437=CARTESIAN_POINT ( 'NONE',  ( -54.20947691318854567, -273.6627369625291522, -199.3366284679518117 ) ) ;
#90438=CARTESIAN_POINT ( 'NONE',  ( 39.70246838695052105, -287.5670368962058205, -271.5512887772176782 ) ) ;
#90439=CARTESIAN_POINT ( 'NONE',  ( -14.96245253393503916, -288.4368304901600482, -344.0708654539153599 ) ) ;
#90440=CARTESIAN_POINT ( 'NONE',  ( -107.4656973267147180, -274.9051788809576351, -243.1501452168379558 ) ) ;
#90441=CARTESIAN_POINT ( 'NONE',  ( -110.2578004204040525, -294.7685807993274807, -253.5304688717324098 ) ) ;
#90442=CARTESIAN_POINT ( 'NONE',  ( 29.61615870820702767, -281.2406369717811572, -308.1630850858723534 ) ) ;
#90444=CARTESIAN_POINT ( 'NONE',  ( -96.33610129740313255, -277.1878192745356841, -224.0303015786622893 ) ) ;
#90446=CARTESIAN_POINT ( 'NONE',  ( -108.7402307614557202, -289.1238630663619347, -287.3723004675085235 ) ) ;
#90449=CARTESIAN_POINT ( 'NONE',  ( -89.29822738331768051, -289.3211376660325413, -216.2012950742297335 ) ) ;
#90450=CARTESIAN_POINT ( 'NONE',  ( -66.10141161950679134, -275.1888895343701620, -202.5113814432587560 ) ) ;
#90451=CARTESIAN_POINT ( 'NONE',  ( 34.04354860159339324, -283.3251045196583391, -297.6146050172361583 ) ) ;
#90452=CARTESIAN_POINT ( 'NONE',  ( -20.93113067675179906, -296.2767230804165592, -195.0114142401944264 ) ) ;
#90453=CARTESIAN_POINT ( 'NONE',  ( -106.9858573769190286, -284.2621611793797456, -292.2401344389542146 ) ) ;
#90454=CARTESIAN_POINT ( 'NONE',  ( -24.51140070544253646, -275.6442507432472553, -197.8469987294978125 ) ) ;
#90455=CARTESIAN_POINT ( 'NONE',  ( 28.00092992438041506, -275.9093325594704993, -237.4530274233429452 ) ) ;
#90456=CARTESIAN_POINT ( 'NONE',  ( -0.1019808792622469984, -284.5569116119880277, -335.4774467391374060 ) ) ;
#90458=CARTESIAN_POINT ( 'NONE',  ( -52.67268509034047241, -296.9097616766705983, -198.6964329503011299 ) ) ;
#90460=CARTESIAN_POINT ( 'NONE',  ( 204.9097360766351130, 294.4826453818760683, -54.00000000002630429 ) ) ;
#90461=CARTESIAN_POINT ( 'NONE',  ( -1.969369272137820870, -294.4300618183150391, -338.7555491472663221 ) ) ;
#90462=CARTESIAN_POINT ( 'NONE',  ( -99.49017384628112382, -287.0933102938046773, -229.0160576099841307 ) ) ;
#90464=CARTESIAN_POINT ( 'NONE',  ( -99.90806341382575795, -281.4094976428775112, -320.2154176792147382 ) ) ;
#90465=CARTESIAN_POINT ( 'NONE',  ( -31.47282331195544458, -276.1771342397307194, -347.0276969494658488 ) ) ;
#90466=CARTESIAN_POINT ( 'NONE',  ( -113.0215390613652460, -288.8341820646413680, -279.6859390279827835 ) ) ;
#90467=CARTESIAN_POINT ( 'NONE',  ( -32.07703169672834775, -284.5046599341272895, -343.8661587566058984 ) ) ;
#90468=CARTESIAN_POINT ( 'NONE',  ( -95.23179281835876964, -279.6696906995564404, -316.4976339776339955 ) ) ;
#90469=CARTESIAN_POINT ( 'NONE',  ( -100.5196209850382019, -286.5495977951537157, -227.2890596849693168 ) ) ;
#90470=CARTESIAN_POINT ( 'NONE',  ( 22.92119638784911118, -282.9427202210016503, -225.6921835737705635 ) ) ;
#90471=CARTESIAN_POINT ( 'NONE',  ( 35.72928442274577776, -275.4112629501662468, -245.9107351557189816 ) ) ;
#90472=CARTESIAN_POINT ( 'NONE',  ( -75.33804700893723805, -277.3776311521315847, -337.3333333275879227 ) ) ;
#90473=CARTESIAN_POINT ( 'NONE',  ( -42.46489358481200327, -297.0374314556101467, -344.6246156608897877 ) ) ;
#90476=CARTESIAN_POINT ( 'NONE',  ( -48.76006227618365330, -296.0479459154993265, -195.4088716011214899 ) ) ;
#90477=CARTESIAN_POINT ( 'NONE',  ( -64.36172741372259054, -276.9220473737363477, -338.2964106327274294 ) ) ;
#90478=CARTESIAN_POINT ( 'NONE',  ( -51.75605163194205005, -298.9516942827281696, -194.9829020043151502 ) ) ;
#90479=CARTESIAN_POINT ( 'NONE',  ( 20.29031449776807960, -288.6644592594607275, -223.9026456087891006 ) ) ;
#90480=CARTESIAN_POINT ( 'NONE',  ( -112.9177906086094936, -298.2064033619323595, -259.7325634386737647 ) ) ;
#90481=CARTESIAN_POINT ( 'NONE',  ( -32.02467138531660851, -296.1915785838982629, -346.7924821553039578 ) ) ;
#90482=CARTESIAN_POINT ( 'NONE',  ( -101.2911949615413647, -293.0744354850784816, -231.4960882580051020 ) ) ;
#90483=CARTESIAN_POINT ( 'NONE',  ( -68.03553479123888792, -277.6480984893867685, -202.0982390200752263 ) ) ;
#90484=CARTESIAN_POINT ( 'NONE',  ( -65.38075117785712109, -281.6028941185841177, -201.4036976774882532 ) ) ;
#90485=CARTESIAN_POINT ( 'NONE',  ( -40.55615258561152103, -296.0912925320236013, -195.9777527788390898 ) ) ;
#90486=CARTESIAN_POINT ( 'NONE',  ( -44.28208289165075939, -284.9993215759203622, -345.8598682605903605 ) ) ;
#90487=CARTESIAN_POINT ( 'NONE',  ( 28.49938087140639098, -286.9073053107481996, -302.5974038332714713 ) ) ;
#90488=CARTESIAN_POINT ( 'NONE',  ( 186.9901108754978054, 262.1367507616976127, -152.9611386112110836 ) ) ;
#90489=CARTESIAN_POINT ( 'NONE',  ( 6.943116152020298415, -286.3404107245024761, -212.2374102784823720 ) ) ;
#90491=CARTESIAN_POINT ( 'NONE',  ( -85.89600774059142907, -284.7865959364761466, -329.7241681159889026 ) ) ;
#90492=CARTESIAN_POINT ( 'NONE',  ( -33.81466304744931506, -298.5898263505375780, -197.2992743959117092 ) ) ;
#90493=CARTESIAN_POINT ( 'NONE',  ( -26.66120766543634701, -284.9799229863747314, -194.4531921616974444 ) ) ;
#90494=CARTESIAN_POINT ( 'NONE',  ( -11.59958383191884224, -281.3204845604748812, -197.9854402697818330 ) ) ;
#90496=CARTESIAN_POINT ( 'NONE',  ( -64.51370615259645547, -281.2240678548217261, -199.0004806361470173 ) ) ;
#90497=CARTESIAN_POINT ( 'NONE',  ( 30.70113632595101549, -281.4191624949866082, -234.2486450573983916 ) ) ;
#90498=CARTESIAN_POINT ( 'NONE',  ( -109.1418805571601069, -282.0523547857346784, -270.3284710469131937 ) ) ;
#90499=CARTESIAN_POINT ( 'NONE',  ( -30.45121505427302822, -124.7187385046102577, -364.4204196855452551 ) ) ;
#90501=CARTESIAN_POINT ( 'NONE',  ( -5.473321563751323282, -278.6321329384867909, -338.0836899838909062 ) ) ;
#90502=CARTESIAN_POINT ( 'NONE',  ( 193.4698978865293100, 279.2676723978439099, -125.7697831199173493 ) ) ;
#90503=CARTESIAN_POINT ( 'NONE',  ( 37.33344107558067293, -279.5491298462316081, -268.5686846150931046 ) ) ;
#90504=CARTESIAN_POINT ( 'NONE',  ( 37.84583692617987083, -295.1685309301496432, -259.0174925633831435 ) ) ;
#90505=CARTESIAN_POINT ( 'NONE',  ( -108.9862823002714691, -295.7085867948225655, -284.9474886127082414 ) ) ;
#90506=CARTESIAN_POINT ( 'NONE',  ( -39.20391299603881663, -291.5370572017369568, -193.4321710414825191 ) ) ;
#90507=CARTESIAN_POINT ( 'NONE',  ( -110.6395987777366372, -271.3322271728258670, -283.6871839692949493 ) ) ;
#90508=CARTESIAN_POINT ( 'NONE',  ( -112.6265387581754567, -294.9584046760650153, -283.7295356724400790 ) ) ;
#90509=CARTESIAN_POINT ( 'NONE',  ( 22.59969361385117637, -286.5473646369430867, -313.4130602447166893 ) ) ;
#90510=CARTESIAN_POINT ( 'NONE',  ( 21.14159985307658118, -294.7785392034865595, -224.6178047424902786 ) ) ;
#90511=CARTESIAN_POINT ( 'NONE',  ( -109.1503233189311572, -286.0730973678907390, -254.6573329654319764 ) ) ;
#90512=CARTESIAN_POINT ( 'NONE',  ( 10.96140137255359193, -293.6428233615162071, -210.6300977006126232 ) ) ;
#90513=CARTESIAN_POINT ( 'NONE',  ( 26.91214494292058390, -282.5186020735537227, -305.1380044889103829 ) ) ;
#90514=CARTESIAN_POINT ( 'NONE',  ( -71.90866226528002869, -294.2938732441011780, -338.7214416260713961 ) ) ;
#90515=CARTESIAN_POINT ( 'NONE',  ( -112.7076064441146457, -291.1665157253328289, -285.3990380602929235 ) ) ;
#90516=CARTESIAN_POINT ( 'NONE',  ( -27.86289646378844154, -292.6616469247202303, -193.9551510633994837 ) ) ;
#90517=CARTESIAN_POINT ( 'NONE',  ( -96.55737201012961179, -290.1217991645716552, -313.0519156803845817 ) ) ;
#90520=CARTESIAN_POINT ( 'NONE',  ( -113.1299716508203801, -298.3858968312070488, -272.4596064290795994 ) ) ;
#90521=CARTESIAN_POINT ( 'NONE',  ( -113.7836448741590232, -271.4189930081095667, -264.6405309598038116 ) ) ;
#90522=CARTESIAN_POINT ( 'NONE',  ( -4.230497036130876687, -279.5584965282023973, -205.0244694356096602 ) ) ;
#90523=ORIENTED_EDGE ( 'NONE', *, *, #31936, .F. ) ;
#90524=CARTESIAN_POINT ( 'NONE',  ( 2.391592923915218272, -274.0773285237768846, -204.4764283617008118 ) ) ;
#90526=CARTESIAN_POINT ( 'NONE',  ( -84.50384236265387017, -295.8692250111691351, -213.6690705701821571 ) ) ;
#90527=CARTESIAN_POINT ( 'NONE',  ( -8.232863205915352367, -278.5273120249084968, -338.6650163409780703 ) ) ;
#90528=CARTESIAN_POINT ( 'NONE',  ( -8.468905047304291500, -272.5735991943565750, -201.9160284759665274 ) ) ;
#90529=CARTESIAN_POINT ( 'NONE',  ( -110.4472800381208373, -297.8501861935719717, -263.2765083089749396 ) ) ;
#90530=CARTESIAN_POINT ( 'NONE',  ( -41.90124506154118222, -299.0730200822998768, -197.1939352843758968 ) ) ;
#90532=CARTESIAN_POINT ( 'NONE',  ( -105.8035841109465736, -298.5864088478954272, -236.9035201173315954 ) ) ;
#90533=CARTESIAN_POINT ( 'NONE',  ( 95.17455889409825431, -297.7070312337581868, -195.2394971372179668 ) ) ;
#90534=CARTESIAN_POINT ( 'NONE',  ( 23.42136893306190615, -293.6399350351919679, -229.7194877680895502 ) ) ;
#90535=CARTESIAN_POINT ( 'NONE',  ( 30.40524502766028903, -291.7426236418784811, -241.4952184992853290 ) ) ;
#90536=CARTESIAN_POINT ( 'NONE',  ( 38.12323504225818738, -276.2320633510027506, -285.3467932484457492 ) ) ;
#90538=CARTESIAN_POINT ( 'NONE',  ( -109.1301048258702906, -272.8971213833867182, -256.8458732120670902 ) ) ;
#90540=CARTESIAN_POINT ( 'NONE',  ( -11.24742307381640849, -284.6938370694468290, -341.1095283698787739 ) ) ;
#90542=CARTESIAN_POINT ( 'NONE',  ( -70.27312709790456324, -282.1618575070084489, -339.4321271594369591 ) ) ;
#90543=CARTESIAN_POINT ( 'NONE',  ( -68.98102638335927850, -276.8059643674052950, -340.4630626115244354 ) ) ;
#90545=CARTESIAN_POINT ( 'NONE',  ( -94.41739525194741134, -283.1037433213924714, -316.1518576435993282 ) ) ;
#90546=CARTESIAN_POINT ( 'NONE',  ( 33.86396058564700695, -279.8645509640809905, -294.6013771361581917 ) ) ;
#90547=CARTESIAN_POINT ( 'NONE',  ( -4.821906802915019163, -275.1900306274544050, -336.3890416430190271 ) ) ;
#90548=CARTESIAN_POINT ( 'NONE',  ( -111.7797188516766198, -280.4293875169361741, -279.9349634603549362 ) ) ;
#90550=CARTESIAN_POINT ( 'NONE',  ( -94.47303263745031643, -271.6419870804418792, -219.9383923306725706 ) ) ;
#90551=CARTESIAN_POINT ( 'NONE',  ( -71.97281133627406291, -279.5090360652539516, -337.0891456231197481 ) ) ;
#90553=CARTESIAN_POINT ( 'NONE',  ( -69.82840687882638520, -285.3966615483934675, -338.5950119462010548 ) ) ;
#90556=CARTESIAN_POINT ( 'NONE',  ( 34.38310171782613622, -285.2673908178722968, -248.2655814507496075 ) ) ;
#90558=CARTESIAN_POINT ( 'NONE',  ( -75.87953643057717557, -294.3737662519613991, -332.8860940508052977 ) ) ;
#90559=CARTESIAN_POINT ( 'NONE',  ( -85.50411400532475170, -287.8656017415780184, -326.9201125168872863 ) ) ;
#90561=CARTESIAN_POINT ( 'NONE',  ( -106.5996002965573695, -294.9276701843219826, -241.5801536071919884 ) ) ;
#90562=CARTESIAN_POINT ( 'NONE',  ( -73.26929873800466453, -284.0648507988596521, -202.9830993872690783 ) ) ;
#90563=CARTESIAN_POINT ( 'NONE',  ( 23.25314589603187798, -283.7330588521203936, -312.4883663038660870 ) ) ;
#90564=CARTESIAN_POINT ( 'NONE',  ( -66.21227798649148610, -281.6647525063432909, -340.6635517949474661 ) ) ;
#90565=CARTESIAN_POINT ( 'NONE',  ( 19.51348556975623083, -288.1995056051616757, -316.1485382993283224 ) ) ;
#90566=CARTESIAN_POINT ( 'NONE',  ( -89.90708202472318078, -280.7175517807921210, -218.7888280785315942 ) ) ;
#90567=CARTESIAN_POINT ( 'NONE',  ( -1.896780215286702154, -281.3373586711661005, -206.3590916116236542 ) ) ;
#90568=CARTESIAN_POINT ( 'NONE',  ( 15.54983676550273053, -290.2889745846089795, -324.1076463553332587 ) ) ;
#90570=CARTESIAN_POINT ( 'NONE',  ( -7.690579524509375986, -274.4300503898912780, -199.2424981971485067 ) ) ;
#90571=CARTESIAN_POINT ( 'NONE',  ( -106.6306356591301636, -292.1669916897665189, -298.2646329065370878 ) ) ;
#90573=CARTESIAN_POINT ( 'NONE',  ( -99.90806341382572953, -299.6948066931273047, -220.5068182859052968 ) ) ;
#90575=CARTESIAN_POINT ( 'NONE',  ( 37.87262138082609653, -273.5624502598165577, -271.1777661500246381 ) ) ;
#90577=CARTESIAN_POINT ( 'NONE',  ( -36.30597713269166604, -293.4392857900434137, -346.5670494187592112 ) ) ;
#90578=CARTESIAN_POINT ( 'NONE',  ( -71.94867088985502335, -272.9307878819382154, -205.9133346863624467 ) ) ;
#90579=CARTESIAN_POINT ( 'NONE',  ( -42.69513748755241522, -290.6408991098892898, -343.9108313187412591 ) ) ;
#90580=CARTESIAN_POINT ( 'NONE',  ( 29.07010127890838191, -283.7503203867120760, -303.1492995913209256 ) ) ;
#90581=CARTESIAN_POINT ( 'NONE',  ( -113.6009320973543169, -292.0380420358455922, -265.5511459457677006 ) ) ;
#90582=CARTESIAN_POINT ( 'NONE',  ( -7.398745630150998842, -293.7518173882294263, -199.9429284146028465 ) ) ;
#90583=CARTESIAN_POINT ( 'NONE',  ( -55.01030098087403530, -291.6518653089868849, -199.5316004888768759 ) ) ;
#90584=CARTESIAN_POINT ( 'NONE',  ( -94.80339294769228786, -287.2184767542982513, -222.1620048122800597 ) ) ;
#90585=CARTESIAN_POINT ( 'NONE',  ( -41.01051860918858694, -280.1738915585690961, -193.4353761973161454 ) ) ;
#90586=CARTESIAN_POINT ( 'NONE',  ( -67.67104348097620914, -293.5268697507071352, -339.5669351673868164 ) ) ;
#90587=CARTESIAN_POINT ( 'NONE',  ( -55.70423773753437757, -283.1155459800356198, -345.1395722125438397 ) ) ;
#90588=CARTESIAN_POINT ( 'NONE',  ( 35.10381599171308409, -277.6234969144568367, -286.6212447235566287 ) ) ;
#90589=CARTESIAN_POINT ( 'NONE',  ( -105.5795714935544112, -286.8376638359844719, -285.9686137636504668 ) ) ;
#90591=CARTESIAN_POINT ( 'NONE',  ( -98.66419258219457333, -276.0915520697607235, -314.8787760645458320 ) ) ;
#90593=CARTESIAN_POINT ( 'NONE',  ( -33.49925342348564783, -282.5101675445274623, -343.3341291046178299 ) ) ;
#90594=CARTESIAN_POINT ( 'NONE',  ( -22.65740913718828153, -281.4410204041606107, -195.1248301900121760 ) ) ;
#90595=CARTESIAN_POINT ( 'NONE',  ( 28.69521240344508328, -287.1224149888095099, -309.5012047962646875 ) ) ;
#90596=CARTESIAN_POINT ( 'NONE',  ( 30.77975472383667821, -294.9275245018964142, -241.2915136975370274 ) ) ;
#90597=CARTESIAN_POINT ( 'NONE',  ( -0.4507878081491541455, -276.1341585071139093, -203.6716920053025319 ) ) ;
#90598=CARTESIAN_POINT ( 'NONE',  ( 2.149019613623236680, -275.8845582162140317, -204.8341668346853908 ) ) ;
#90599=CARTESIAN_POINT ( 'NONE',  ( -87.09708192572611551, -277.6021384487344790, -323.7783622643488002 ) ) ;
#90600=CARTESIAN_POINT ( 'NONE',  ( -106.4651649713362218, -298.9273471198818584, -241.6910110428851226 ) ) ;
#90601=CARTESIAN_POINT ( 'NONE',  ( -74.44298135506785741, -283.5574047911027833, -205.3576201718144034 ) ) ;
#90602=CARTESIAN_POINT ( 'NONE',  ( 13.26776739764922297, -292.4043044654659411, -212.3574449246964662 ) ) ;
#90603=CARTESIAN_POINT ( 'NONE',  ( 20.89097088326920471, -289.8212973518486706, -319.5078009258397742 ) ) ;
#90604=CARTESIAN_POINT ( 'NONE',  ( 35.93072163279381925, -292.4420104958599040, -268.0420056553431323 ) ) ;
#90606=CARTESIAN_POINT ( 'NONE',  ( -69.35957396144178233, -290.2138235857514701, -200.9677691882640431 ) ) ;
#90607=CARTESIAN_POINT ( 'NONE',  ( -33.50308118302822891, -291.7684830894787069, -197.4284433137697761 ) ) ;
#90609=CARTESIAN_POINT ( 'NONE',  ( -3.185999573392908957, -289.6913388354190033, -339.0406772653464031 ) ) ;
#90610=CARTESIAN_POINT ( 'NONE',  ( -81.30399101819510577, -279.7692269770939220, -211.9932115196273799 ) ) ;
#90611=CARTESIAN_POINT ( 'NONE',  ( -68.04103870623133332, -296.5789054304839851, -200.0262277653163494 ) ) ;
#90612=CARTESIAN_POINT ( 'NONE',  ( -87.68947464013822923, -286.0221398584377539, -212.1664879785889752 ) ) ;
#90613=CARTESIAN_POINT ( 'NONE',  ( -4.786748280962233260, -286.8025829718178557, -200.6049755872068374 ) ) ;
#90614=CARTESIAN_POINT ( 'NONE',  ( -106.1922471466907183, -284.5600154893914464, -294.8363354118778261 ) ) ;
#90615=CARTESIAN_POINT ( 'NONE',  ( 203.3290562182569090, 295.9433822784110362, -54.00000000004157386 ) ) ;
#90616=CARTESIAN_POINT ( 'NONE',  ( -100.5277185204516144, -246.4223321106570097, -332.7819595289345216 ) ) ;
#90617=CARTESIAN_POINT ( 'NONE',  ( 137.9338102360727873, 178.6954944670252416, -238.2672434279379843 ) ) ;
#90618=CARTESIAN_POINT ( 'NONE',  ( 33.99349039586270038, -274.5348307297093697, -254.0603081086666464 ) ) ;
#90619=CARTESIAN_POINT ( 'NONE',  ( -9.885297577637768285, -275.6052940316844797, -338.3480584340046562 ) ) ;
#90620=CARTESIAN_POINT ( 'NONE',  ( -93.61345767255416206, -296.7763583323657031, -217.8142208377114457 ) ) ;
#90621=CARTESIAN_POINT ( 'NONE',  ( 85.86301894190751227, 81.15251262249802267, -299.4358512761199336 ) ) ;
#90622=CARTESIAN_POINT ( 'NONE',  ( 35.26728156765977928, -273.9296478136211022, -246.0852129532705703 ) ) ;
#90623=CARTESIAN_POINT ( 'NONE',  ( -85.99290297156427698, -275.1275707684375220, -214.5161435434588100 ) ) ;
#90625=CARTESIAN_POINT ( 'NONE',  ( -81.08540120362570747, -274.5531893405452593, -207.3048453682714580 ) ) ;
#90626=CARTESIAN_POINT ( 'NONE',  ( -107.8128992308467815, -291.2990398897558748, -251.0790398058898631 ) ) ;
#90627=CARTESIAN_POINT ( 'NONE',  ( -50.42993694010502992, -296.0178825118061923, -346.1305805619630860 ) ) ;
#90628=CARTESIAN_POINT ( 'NONE',  ( -112.2159187317890598, -297.2660806873803381, -252.6586240328183521 ) ) ;
#90629=CARTESIAN_POINT ( 'NONE',  ( -86.48840921147282756, -295.9246126122980627, -324.3389003634646315 ) ) ;
#90631=CARTESIAN_POINT ( 'NONE',  ( -42.67957362113180153, -279.0391638687532918, -345.7323413049605847 ) ) ;
#90634=CARTESIAN_POINT ( 'NONE',  ( 38.19546491524776144, -280.8768524322094891, -255.7438815600982025 ) ) ;
#90635=CARTESIAN_POINT ( 'NONE',  ( 9.824706139981804753, -277.3249706530182834, -326.3855641391881477 ) ) ;
#90636=CARTESIAN_POINT ( 'NONE',  ( 21.86572908666779824, -277.9592877654428662, -318.0100010161548880 ) ) ;
#90637=CARTESIAN_POINT ( 'NONE',  ( -106.0861757196606163, -276.1680286674200602, -301.3524653305345282 ) ) ;
#90638=CARTESIAN_POINT ( 'NONE',  ( -27.28790972808698001, -274.6755835064429903, -197.9436809192020803 ) ) ;
#90639=CARTESIAN_POINT ( 'NONE',  ( -80.05542733467437699, -296.0359304892675141, -210.4368956361018093 ) ) ;
#90642=CARTESIAN_POINT ( 'NONE',  ( -107.2277311223854070, -278.9981054427363460, -249.2674536168235875 ) ) ;
#90643=CARTESIAN_POINT ( 'NONE',  ( -45.98678922299930605, -287.8442927162407727, -346.4307498323549339 ) ) ;
#90644=CARTESIAN_POINT ( 'NONE',  ( -32.82907011243004547, -276.1091532367080390, -195.4841864206673847 ) ) ;
#90646=CARTESIAN_POINT ( 'NONE',  ( -96.69559085280752697, -289.1524431895654175, -313.1363138688400909 ) ) ;
#90647=CARTESIAN_POINT ( 'NONE',  ( -89.81062465253063465, -284.6836706174646565, -214.0719371500587442 ) ) ;
#90648=CARTESIAN_POINT ( 'NONE',  ( 33.92926937936289278, -280.0522227695563515, -290.3216520527920466 ) ) ;
#90649=CARTESIAN_POINT ( 'NONE',  ( 32.78734996933208379, -280.4221407947374018, -292.8269739511292755 ) ) ;
#90650=CARTESIAN_POINT ( 'NONE',  ( -108.7290556674159063, -282.9078703479744945, -249.0837395250946713 ) ) ;
#90652=CARTESIAN_POINT ( 'NONE',  ( -69.51293540009807259, -287.6289154997058972, -202.5975507336678163 ) ) ;
#90653=CARTESIAN_POINT ( 'NONE',  ( -103.4822045126110481, -279.3276377534990615, -302.2994821243185015 ) ) ;
#90655=CARTESIAN_POINT ( 'NONE',  ( -44.72615378725276969, -293.9589824281899268, -195.6739853190973975 ) ) ;
#90656=CARTESIAN_POINT ( 'NONE',  ( -112.2339107445989868, -276.9548691370670213, -257.5107948838872858 ) ) ;
#90658=CARTESIAN_POINT ( 'NONE',  ( 19.26578866550989133, -276.8577630935376988, -316.6354122796417982 ) ) ;
#90659=CARTESIAN_POINT ( 'NONE',  ( -4.930710786768611520, -284.6265849785726232, -338.1952929343584060 ) ) ;
#90661=CARTESIAN_POINT ( 'NONE',  ( -90.56650167772804139, -291.7187488390284216, -324.0670995159550216 ) ) ;
#90662=CARTESIAN_POINT ( 'NONE',  ( -75.10123183301142546, -293.5550138477503879, -335.1772404801290577 ) ) ;
#90663=CARTESIAN_POINT ( 'NONE',  ( 35.69874235161989873, -286.4465967501391219, -246.3318718969451311 ) ) ;
#90664=CARTESIAN_POINT ( 'NONE',  ( -49.80398252576205920, -290.2905506021631368, -197.5690644006636774 ) ) ;
#90666=CARTESIAN_POINT ( 'NONE',  ( 34.64424301569840736, -274.4310025422716990, -285.1688007543081653 ) ) ;
#90667=CARTESIAN_POINT ( 'NONE',  ( -35.64575197263904016, -293.1702674211743442, -344.5896546003434651 ) ) ;
#90670=CARTESIAN_POINT ( 'NONE',  ( -112.9762366047404640, -289.1644397743135642, -259.8693321595174552 ) ) ;
#90671=CARTESIAN_POINT ( 'NONE',  ( -75.14723633963060934, -287.1393933818288815, -206.9798759082806896 ) ) ;
#90672=CARTESIAN_POINT ( 'NONE',  ( -71.47167865511831053, -287.7366007749833443, -338.2516076156232998 ) ) ;
#90673=CARTESIAN_POINT ( 'NONE',  ( -104.0270410264673728, -286.3957068942892192, -239.1204850148393177 ) ) ;
#90675=CARTESIAN_POINT ( 'NONE',  ( -95.09080413602785598, -285.9866801744764189, -225.4225942282864423 ) ) ;
#90676=CARTESIAN_POINT ( 'NONE',  ( 12.17821917378289953, -294.7171054700545483, -213.5616074885234354 ) ) ;
#90677=CARTESIAN_POINT ( 'NONE',  ( -41.33329328226338362, -275.1818595130561107, -345.8285784664917060 ) ) ;
#90678=CARTESIAN_POINT ( 'NONE',  ( 29.07984607417623835, -276.3920240203173080, -309.2702748940043875 ) ) ;
#90679=CARTESIAN_POINT ( 'NONE',  ( 21.99279681067072900, -290.9941651548755885, -223.5565506714850414 ) ) ;
#90680=CARTESIAN_POINT ( 'NONE',  ( -93.07375337715214414, -279.2792445185638712, -217.1536065092782906 ) ) ;
#90681=CARTESIAN_POINT ( 'NONE',  ( -111.8828994258877430, -298.4813300197060357, -274.2925817380099716 ) ) ;
#90684=CARTESIAN_POINT ( 'NONE',  ( -111.5152681033728612, -276.6524956580881849, -273.3855669416655019 ) ) ;
#90685=CARTESIAN_POINT ( 'NONE',  ( 37.62000210017881585, -279.5827599649646800, -272.7577499571896169 ) ) ;
#90687=CARTESIAN_POINT ( 'NONE',  ( 36.91265796786614573, -274.2545288238475223, -287.9956782465559399 ) ) ;
#90688=CARTESIAN_POINT ( 'NONE',  ( 6.490727046354843210, -295.9647838861012588, -329.6651332146280993 ) ) ;
#90689=CARTESIAN_POINT ( 'NONE',  ( -33.08968521958203723, -281.9201386677901269, -346.9471255576982003 ) ) ;
#90690=CARTESIAN_POINT ( 'NONE',  ( -88.65819797007746672, -296.7348767808570074, -322.6820201918375233 ) ) ;
#90691=CARTESIAN_POINT ( 'NONE',  ( -67.99535505441080829, -298.9733638128169559, -200.2072329143113905 ) ) ;
#90692=CARTESIAN_POINT ( 'NONE',  ( -5.294946954141301454, -274.1526001175590181, -204.7340811125050095 ) ) ;
#90693=CARTESIAN_POINT ( 'NONE',  ( -25.10726373508821396, -294.2081860196391290, -196.3128317803379446 ) ) ;
#90694=CARTESIAN_POINT ( 'NONE',  ( 36.38600856691606111, -287.9980934139662168, -292.6155855646658210 ) ) ;
#90695=CARTESIAN_POINT ( 'NONE',  ( 35.30228972421073763, -273.9666682000668061, -291.9279064809528563 ) ) ;
#90696=CARTESIAN_POINT ( 'NONE',  ( -46.02787954747933696, -288.9926015983626257, -346.9227429523101023 ) ) ;
#90697=CARTESIAN_POINT ( 'NONE',  ( 34.23810733270660478, -286.8152198767577943, -285.9034150297784436 ) ) ;
#90698=CARTESIAN_POINT ( 'NONE',  ( -39.13758790572180146, -290.0294877941399818, -195.3699211357650540 ) ) ;
#90701=CARTESIAN_POINT ( 'NONE',  ( 12.19292191415735971, -287.8484076537902183, -324.1356281857199519 ) ) ;
#90703=CARTESIAN_POINT ( 'NONE',  ( -71.62287469123025119, -284.4352618367339005, -339.0460601790132387 ) ) ;
#90704=CARTESIAN_POINT ( 'NONE',  ( 38.99349840474387463, -292.5030567905028533, -261.7642130439592734 ) ) ;
#90705=CARTESIAN_POINT ( 'NONE',  ( -25.53980054998473648, -281.8002742272543628, -195.0806053637984121 ) ) ;
#90706=CARTESIAN_POINT ( 'NONE',  ( -50.86899104264909965, -281.1979495101255111, -195.0596527109729550 ) ) ;
#90707=CARTESIAN_POINT ( 'NONE',  ( -71.41076191019858754, -283.3486884180255174, -334.9234834427126657 ) ) ;
#90708=CARTESIAN_POINT ( 'NONE',  ( -67.58645676448941231, -279.4491100240194328, -338.9924180400056457 ) ) ;
#90709=CARTESIAN_POINT ( 'NONE',  ( -110.8131257326467392, -296.8436739640969790, -247.1420255719417298 ) ) ;
#90710=CARTESIAN_POINT ( 'NONE',  ( -32.67634471788182537, -275.4273242342445087, -197.0035825727832446 ) ) ;
#90711=CARTESIAN_POINT ( 'NONE',  ( -111.7646678862558929, -288.4898831002248585, -276.7460579482406047 ) ) ;
#90712=CARTESIAN_POINT ( 'NONE',  ( -81.29659581834329174, -272.2346935961606960, -211.5172749958831275 ) ) ;
#90716=CARTESIAN_POINT ( 'NONE',  ( -111.7494130062512312, -286.5006740938570147, -268.1687541312248300 ) ) ;
#90717=CARTESIAN_POINT ( 'NONE',  ( 31.95662831818015093, -295.0559047529468444, -303.3366583851507130 ) ) ;
#90718=CARTESIAN_POINT ( 'NONE',  ( -89.74170372891182978, -285.9402786022944269, -219.3165910058665418 ) ) ;
#90719=CARTESIAN_POINT ( 'NONE',  ( 32.79990346686290792, -275.0102467585803652, -301.5536757076124559 ) ) ;
#90720=CARTESIAN_POINT ( 'NONE',  ( -112.8264954240849676, -291.3881973638704608, -255.6173880199340545 ) ) ;
#90721=CARTESIAN_POINT ( 'NONE',  ( -35.15968300279987346, -284.2188319458764454, -194.6148093390386009 ) ) ;
#90723=CARTESIAN_POINT ( 'NONE',  ( -67.01121706702680569, -292.0070216581106024, -199.3296879239660768 ) ) ;
#90724=CARTESIAN_POINT ( 'NONE',  ( -73.55176158966020239, -289.8801298503398129, -333.7862494643336504 ) ) ;
#90727=CARTESIAN_POINT ( 'NONE',  ( -110.7271127053023747, -271.1905260033421428, -283.6752375529766255 ) ) ;
#90728=CIRCLE ( 'NONE', #42363, 6.649382010133625620 ) ;
#90729=CARTESIAN_POINT ( 'NONE',  ( -3.185662161419823057, -284.1294238190711212, -338.6110628531907309 ) ) ;
#90730=CARTESIAN_POINT ( 'NONE',  ( -85.28047601435909542, -282.9094976428775681, -210.1954327657594206 ) ) ;
#90732=CARTESIAN_POINT ( 'NONE',  ( 14.13197469526531869, -281.2290757296504466, -322.6311112145170341 ) ) ;
#90733=CARTESIAN_POINT ( 'NONE',  ( -70.29581879405932909, -277.1413115772413676, -339.9440097967894872 ) ) ;
#90734=CARTESIAN_POINT ( 'NONE',  ( -24.58837989201014196, -282.2154531742766608, -196.6225171904349338 ) ) ;
#90735=CARTESIAN_POINT ( 'NONE',  ( -28.99282367148100903, -125.6822456004873771, -362.4878069686170079 ) ) ;
#90737=CARTESIAN_POINT ( 'NONE',  ( 37.41203481182020596, -279.9266348538377542, -254.4717227220314442 ) ) ;
#90738=CARTESIAN_POINT ( 'NONE',  ( -57.82199640242539118, -283.8065939204187202, -198.5270754086298268 ) ) ;
#90739=CARTESIAN_POINT ( 'NONE',  ( -96.85772876603391524, -275.0498151047976307, -223.4767088475412891 ) ) ;
#90740=CARTESIAN_POINT ( 'NONE',  ( -106.9259586923700738, -296.7474464306404798, -292.7963462226406364 ) ) ;
#90742=CARTESIAN_POINT ( 'NONE',  ( 15.23997291625055972, -291.4984240644922124, -218.9422159366309302 ) ) ;
#90743=CARTESIAN_POINT ( 'NONE',  ( -65.05058793322571375, -278.0560987127101953, -342.1496786930522944 ) ) ;
#90744=CARTESIAN_POINT ( 'NONE',  ( 13.49665661008067197, -274.7884575658887343, -217.9735098661038819 ) ) ;
#90745=CARTESIAN_POINT ( 'NONE',  ( 38.19007794046916615, -274.3047475889360953, -257.0028189701606038 ) ) ;
#90746=DIRECTION ( 'NONE',  ( 0.000000000000000000, 0.000000000000000000, -1.000000000000000000 ) ) ;
#90747=CARTESIAN_POINT ( 'NONE',  ( 15.92346366696724758, -272.8062822572314303, -217.4885609906349089 ) ) ;
#90751=CARTESIAN_POINT ( 'NONE',  ( -40.23284258655100842, -284.1690195968155876, -343.6131989739774326 ) ) ;
#90752=CARTESIAN_POINT ( 'NONE',  ( 27.45281009266694028, -283.8389541093177399, -310.1552793963434738 ) ) ;
#90753=CARTESIAN_POINT ( 'NONE',  ( -91.59130234939324566, -284.6022041161181733, -221.2880414379674505 ) ) ;
#90754=CARTESIAN_POINT ( 'NONE',  ( -37.83534143752670076, -275.4582703718180028, -344.1720588528639269 ) ) ;
#90755=CARTESIAN_POINT ( 'NONE',  ( 25.18338072479433620, -283.9580495583956576, -310.4741544580930963 ) ) ;
#90756=CARTESIAN_POINT ( 'NONE',  ( -95.00757145578261031, -276.3899587625733716, -316.2654287131900332 ) ) ;
#90758=CARTESIAN_POINT ( 'NONE',  ( 34.92807391409401419, -276.4692673562082632, -257.9859943910513493 ) ) ;
#90760=CARTESIAN_POINT ( 'NONE',  ( -39.59279386983942572, -280.8274204208516380, -193.5425520394794603 ) ) ;
#90764=CARTESIAN_POINT ( 'NONE',  ( -40.78444846782597466, -287.8698272199731036, -194.6232190237568602 ) ) ;
#90765=CARTESIAN_POINT ( 'NONE',  ( -98.87464204118074917, -295.2017193826217181, -310.0304370559154563 ) ) ;
#90767=CARTESIAN_POINT ( 'NONE',  ( -110.6871379944550284, -289.6080601826063798, -293.6383752179008866 ) ) ;
#90768=CARTESIAN_POINT ( 'NONE',  ( 32.40479769056452852, -285.8176067488831791, -246.8919688947097484 ) ) ;
#90769=CARTESIAN_POINT ( 'NONE',  ( -109.9369931501766473, -288.6035623757123290, -284.8446897221598419 ) ) ;
#90770=CARTESIAN_POINT ( 'NONE',  ( -109.3213669527072796, -285.9455691458234696, -256.0063950772644148 ) ) ;
#90771=CARTESIAN_POINT ( 'NONE',  ( 35.69330733689766788, -273.3323524578737533, -253.2497194818602679 ) ) ;
#90772=CARTESIAN_POINT ( 'NONE',  ( 15.75648205511122413, -285.1888796384633338, -215.7074496420666492 ) ) ;
#90773=CARTESIAN_POINT ( 'NONE',  ( -94.07536742764946780, -299.2332506693597338, -221.2296079597851701 ) ) ;
#90774=CARTESIAN_POINT ( 'NONE',  ( 35.60398651599691533, -285.3195529151811911, -252.2239949935032257 ) ) ;
#90776=CARTESIAN_POINT ( 'NONE',  ( -59.81720391746119958, -280.6950983122616776, -200.6064174696220732 ) ) ;
#90777=CARTESIAN_POINT ( 'NONE',  ( -40.24189749623339196, -291.0886579452007936, -345.4845886921014539 ) ) ;
#90780=CARTESIAN_POINT ( 'NONE',  ( -47.41494026100687620, -297.0993814537765729, -345.2466575045077093 ) ) ;
#90781=CARTESIAN_POINT ( 'NONE',  ( -95.47504139763903197, -277.2049161283542276, -222.9742496968694070 ) ) ;
#90782=CARTESIAN_POINT ( 'NONE',  ( 37.26761126129164836, -292.5189842737098616, -251.9869656163303375 ) ) ;
#90783=CARTESIAN_POINT ( 'NONE',  ( -102.1797782835470372, -294.4761343281002155, -305.6097212797882889 ) ) ;
#90784=CARTESIAN_POINT ( 'NONE',  ( 22.52487147336448103, -279.6455000491359328, -227.7320541480066822 ) ) ;
#90785=CARTESIAN_POINT ( 'NONE',  ( 24.25741404626410613, -273.0617666028388726, -228.5427492967688465 ) ) ;
#90786=CARTESIAN_POINT ( 'NONE',  ( 32.26272471197889047, -294.5541223951385064, -246.6132427903760629 ) ) ;
#90787=CARTESIAN_POINT ( 'NONE',  ( -4.771743288812468897, -297.1233781216987495, -337.9199732462171255 ) ) ;
#90788=CARTESIAN_POINT ( 'NONE',  ( -98.52482178799844803, -295.6443190632586493, -224.7396090861023197 ) ) ;
#90789=CARTESIAN_POINT ( 'NONE',  ( 1.235417138314658825, -292.7842079968534676, -335.8269872350154515 ) ) ;
#90790=CARTESIAN_POINT ( 'NONE',  ( -97.25155038459429591, -292.5706966546655963, -227.5410149624957228 ) ) ;
#90792=CARTESIAN_POINT ( 'NONE',  ( -32.15602269518463174, -292.9220355325602441, -197.3710042110249674 ) ) ;
#90795=CARTESIAN_POINT ( 'NONE',  ( -75.93759716164696272, -281.5845770773004801, -335.1422854697101457 ) ) ;
#90796=CARTESIAN_POINT ( 'NONE',  ( 32.75017600945747631, -293.8225269863071958, -290.8052846791266575 ) ) ;
#90797=CARTESIAN_POINT ( 'NONE',  ( 29.76189961588162802, -282.0433402970852512, -308.2336156541696255 ) ) ;
#90798=CARTESIAN_POINT ( 'NONE',  ( -27.37904345720521349, -282.5957119380627773, -346.7459110438595076 ) ) ;
#90799=CARTESIAN_POINT ( 'NONE',  ( -51.11323504701555009, -287.2282702317662597, -343.9693374711361002 ) ) ;
#90801=CARTESIAN_POINT ( 'NONE',  ( 36.86950565664233181, -280.2568201587477574, -288.1764287928633621 ) ) ;
#90802=CARTESIAN_POINT ( 'NONE',  ( 39.29470688452499871, -286.5234531919795700, -274.4203385729160232 ) ) ;
#90804=CARTESIAN_POINT ( 'NONE',  ( 35.26662907435790117, -294.9790120047310324, -257.0822072083031458 ) ) ;
#90805=CARTESIAN_POINT ( 'NONE',  ( 7.906858141154913255, -277.8730543295356483, -331.9991500484283620 ) ) ;
#90806=CARTESIAN_POINT ( 'NONE',  ( -49.14114707759480893, -279.5643449837300523, -198.2996127361045922 ) ) ;
#90807=CARTESIAN_POINT ( 'NONE',  ( 15.43662031107284527, -292.9399943472093355, -214.2214419023893015 ) ) ;
#90808=CARTESIAN_POINT ( 'NONE',  ( -95.18405559082212619, -281.9647369262138454, -318.9977694731877591 ) ) ;
#90809=CARTESIAN_POINT ( 'NONE',  ( 27.70098935140995877, -292.1546597211358289, -236.7031769777707382 ) ) ;
#90810=CARTESIAN_POINT ( 'NONE',  ( -72.32446760326256197, -295.5895106967657284, -203.9622226827561349 ) ) ;
#90813=CARTESIAN_POINT ( 'NONE',  ( 25.84274323658424066, -293.5626646024749675, -307.0451002940258149 ) ) ;
#90815=CARTESIAN_POINT ( 'NONE',  ( -105.5795714935544112, -294.2666405000204009, -254.7536222014695397 ) ) ;
#90816=CARTESIAN_POINT ( 'NONE',  ( -43.25962040804878939, -297.0380362544216837, -193.7718148774431768 ) ) ;
#90817=CARTESIAN_POINT ( 'NONE',  ( 24.90182803548134416, -280.2719941749095938, -313.5817110121290057 ) ) ;
#90818=CARTESIAN_POINT ( 'NONE',  ( 23.45926181923605114, -288.2439211521247557, -223.9010684759691685 ) ) ;
#90819=CARTESIAN_POINT ( 'NONE',  ( -53.41059323400035197, -289.0973876626331958, -341.5706024550187294 ) ) ;
#90820=CARTESIAN_POINT ( 'NONE',  ( -43.24349816381648992, -278.6481559529793799, -343.8177482659192492 ) ) ;
#90821=CARTESIAN_POINT ( 'NONE',  ( -111.6861101016002067, -294.6657313476734430, -263.1154739724864271 ) ) ;
#90822=CARTESIAN_POINT ( 'NONE',  ( -110.3774713696544012, -274.2950787127233525, -259.4179901304113400 ) ) ;
#90823=CARTESIAN_POINT ( 'NONE',  ( -94.77328336420495702, -276.7049539764182100, -316.0839746052255919 ) ) ;
#90824=ORIENTED_EDGE ( 'NONE', *, *, #75312, .T. ) ;
#90825=CARTESIAN_POINT ( 'NONE',  ( -33.33159068575541539, -297.7677945479111372, -193.3824812397034236 ) ) ;
#90826=CARTESIAN_POINT ( 'NONE',  ( -78.95963072396740756, -291.5377859905910896, -332.1423800828387130 ) ) ;
#90827=CARTESIAN_POINT ( 'NONE',  ( 16.90561464842478046, -294.4088868646498440, -216.7735773249501676 ) ) ;
#90830=CARTESIAN_POINT ( 'NONE',  ( -94.37564041733163833, -291.8491158251868001, -224.6135265382596060 ) ) ;
#90832=CARTESIAN_POINT ( 'NONE',  ( -114.1314867415316030, -297.1412005554776670, -275.3410497286744203 ) ) ;
#90833=CARTESIAN_POINT ( 'NONE',  ( -76.51008214538381935, -289.6740885983111298, -205.4458354417788541 ) ) ;
#90834=CARTESIAN_POINT ( 'NONE',  ( 30.76082294611260082, -299.2162576857911063, -193.3785011460888654 ) ) ;
#90837=CARTESIAN_POINT ( 'NONE',  ( -102.6327255629189352, -292.5935519350809955, -230.7650273092966984 ) ) ;
#90838=CARTESIAN_POINT ( 'NONE',  ( 25.22466315766300227, -296.6948066931273047, -320.2154176792147382 ) ) ;
#90839=CARTESIAN_POINT ( 'NONE',  ( -69.58743246951203787, -287.6268861102293499, -202.8174215943278398 ) ) ;
#90840=CARTESIAN_POINT ( 'NONE',  ( -43.15570500971156065, -287.6989405396924440, -346.5503799566787961 ) ) ;
#90841=CARTESIAN_POINT ( 'NONE',  ( -46.37546007465596887, -271.9370851207518740, -196.0750519516181782 ) ) ;
#90842=CARTESIAN_POINT ( 'NONE',  ( -62.53968889775161699, -275.6418600410761996, -200.3155930780314122 ) ) ;
#90843=CARTESIAN_POINT ( 'NONE',  ( -96.93554681567800912, -288.0177496538732953, -314.9905557626221935 ) ) ;
#90844=CARTESIAN_POINT ( 'NONE',  ( -112.0768018849169749, -280.2543386846155613, -282.8098145750989261 ) ) ;
#90846=CARTESIAN_POINT ( 'NONE',  ( 15.25938121658180435, -280.8206030763413423, -219.6714554728410178 ) ) ;
#90847=CARTESIAN_POINT ( 'NONE',  ( 11.37992084315340513, -280.0977708659839891, -215.8625279289563537 ) ) ;
#90848=CARTESIAN_POINT ( 'NONE',  ( 39.32149395882056808, -276.6059440806427574, -268.3002489213911872 ) ) ;
#90849=CARTESIAN_POINT ( 'NONE',  ( 8.322209442178680305, -279.4561546196263748, -208.7905692509054063 ) ) ;
#90850=CARTESIAN_POINT ( 'NONE',  ( -90.35769054958068125, -228.8493742786694440, -345.0038117470676866 ) ) ;
#90851=CARTESIAN_POINT ( 'NONE',  ( -2.674560634404023585, -275.4404502270335797, -201.8555152988813290 ) ) ;
#90852=CARTESIAN_POINT ( 'NONE',  ( -94.57934650329326587, -274.7617333585757251, -219.8976699130175803 ) ) ;
#90854=CARTESIAN_POINT ( 'NONE',  ( -106.6662871844225293, -299.4805209788416391, -237.0123917617630980 ) ) ;
#90856=CARTESIAN_POINT ( 'NONE',  ( 104.1717476309105166, -299.5541904835127980, -197.7570935515975350 ) ) ;
#90857=CARTESIAN_POINT ( 'NONE',  ( 17.11104174832909663, -287.9317725444258258, -221.2595437054770002 ) ) ;
#90858=CARTESIAN_POINT ( 'NONE',  ( 19.51344350397417315, -288.6195272223346819, -219.8705124428961142 ) ) ;
#90859=CARTESIAN_POINT ( 'NONE',  ( -109.8916939146382816, -289.7826226818954183, -279.3272247022040347 ) ) ;
#90860=CARTESIAN_POINT ( 'NONE',  ( -49.32894999990031693, -285.4110634945222387, -194.3085259379780325 ) ) ;
#90862=CARTESIAN_POINT ( 'NONE',  ( -23.93999431430018987, -281.2779635836222383, -342.9340791629549585 ) ) ;
#90863=CARTESIAN_POINT ( 'NONE',  ( 35.22304619055572772, -289.6164337645341220, -286.0804274914435155 ) ) ;
#90864=CARTESIAN_POINT ( 'NONE',  ( -36.20204257885875165, -281.5174831966717193, -344.0456410188638188 ) ) ;
#90865=CARTESIAN_POINT ( 'NONE',  ( -109.9769243189216468, -279.7206180160303006, -281.5578891740382801 ) ) ;
#90866=CARTESIAN_POINT ( 'NONE',  ( 17.48555786604638485, -276.7336534365163061, -318.6703679497812800 ) ) ;
#90867=CARTESIAN_POINT ( 'NONE',  ( -95.16869143061067859, -288.6645133080202754, -320.6010204133932007 ) ) ;
#90868=CARTESIAN_POINT ( 'NONE',  ( -107.7822010621069495, -285.7486361629958651, -239.5312209689940630 ) ) ;
#90869=CARTESIAN_POINT ( 'NONE',  ( -93.87878023363248303, -285.7562238965024335, -218.0998392268156181 ) ) ;
#90870=CARTESIAN_POINT ( 'NONE',  ( 19.35338267844834803, -282.3696860666522070, -316.3663370656909706 ) ) ;
#90873=CARTESIAN_POINT ( 'NONE',  ( -96.51397491429513309, -293.0566706825098322, -223.0436013349047926 ) ) ;
#90874=CARTESIAN_POINT ( 'NONE',  ( -76.89984542897843767, -290.2192425981789370, -204.8137575633448932 ) ) ;
#90875=CARTESIAN_POINT ( 'NONE',  ( 34.06585772786585409, -274.3964337372952969, -254.0455763294952476 ) ) ;
#90877=CARTESIAN_POINT ( 'NONE',  ( -70.77106948570759926, -294.8300760074432105, -339.6272524197201506 ) ) ;
#90878=CARTESIAN_POINT ( 'NONE',  ( -75.32048722799150653, -290.0161769980778672, -207.1484076620558596 ) ) ;
#90879=CARTESIAN_POINT ( 'NONE',  ( -2.688886289797828510, -292.8271885715830081, -335.7610912881140166 ) ) ;
#90880=CARTESIAN_POINT ( 'NONE',  ( -103.1949725731118548, -291.3204147236751282, -302.7721810921186147 ) ) ;
#90882=CARTESIAN_POINT ( 'NONE',  ( -62.07930559428666584, -291.3738143728981527, -341.2189367471137302 ) ) ;
#90883=CARTESIAN_POINT ( 'NONE',  ( 12.09238538302695964, -290.7376934807101634, -213.7369216224489605 ) ) ;
#90884=CARTESIAN_POINT ( 'NONE',  ( -39.54149075581725725, -297.0799038051904972, -345.3415077715028474 ) ) ;
#90885=CARTESIAN_POINT ( 'NONE',  ( -65.19377429677207658, -286.6204118655235220, -202.5747882988739832 ) ) ;
#90886=CARTESIAN_POINT ( 'NONE',  ( -39.04025641984931383, -297.0735797031048264, -345.5085952295960965 ) ) ;
#90887=CARTESIAN_POINT ( 'NONE',  ( 37.29158456131943922, -277.3990652573534135, -259.9553686505958581 ) ) ;
#90888=CARTESIAN_POINT ( 'NONE',  ( -48.45164520234993688, -275.9853577955981905, -346.2077291237597478 ) ) ;
#90889=CARTESIAN_POINT ( 'NONE',  ( -9.173577916030799528, -297.5935730249259450, -193.5263149346576199 ) ) ;
#90890=CARTESIAN_POINT ( 'NONE',  ( 14.42427113825025131, -274.5522663346434911, -323.3310379801695831 ) ) ;
#90891=CARTESIAN_POINT ( 'NONE',  ( -38.34925143423605931, -278.1192762904393589, -195.9152880886290973 ) ) ;
#90892=CARTESIAN_POINT ( 'NONE',  ( -89.53526027299699308, -274.5011211024885256, -218.7572151846734698 ) ) ;
#90894=CARTESIAN_POINT ( 'NONE',  ( -35.82159879687392845, -298.8744944963281682, -197.1994263732142656 ) ) ;
#90896=CARTESIAN_POINT ( 'NONE',  ( -2.582332419602012319, -286.6148377780398278, -337.2206211381853223 ) ) ;
#90897=CARTESIAN_POINT ( 'NONE',  ( 34.37389770579854087, -275.2056226547447864, -256.7275919583309474 ) ) ;
#90898=CARTESIAN_POINT ( 'NONE',  ( 12.41582732293890246, -288.3809887253688089, -329.1249543273815448 ) ) ;
#90899=CARTESIAN_POINT ( 'NONE',  ( -20.50516476239022978, -288.5084943617802082, -345.5308504021601834 ) ) ;
#90900=CARTESIAN_POINT ( 'NONE',  ( -109.2230788738129519, -298.2411465925107450, -293.0200560701889003 ) ) ;
#90901=CARTESIAN_POINT ( 'NONE',  ( 25.96493789897412086, -292.0908665092681531, -310.3620141877276524 ) ) ;
#90902=CARTESIAN_POINT ( 'NONE',  ( 24.97033517346224940, -281.3469747147189537, -315.3430872376789011 ) ) ;
#90904=CARTESIAN_POINT ( 'NONE',  ( -64.55037024555267067, -277.6969516674083707, -200.4157805965516559 ) ) ;
#90906=CARTESIAN_POINT ( 'NONE',  ( -50.83946396662989287, -288.0232270138000104, -342.5583561058506348 ) ) ;
#90909=CARTESIAN_POINT ( 'NONE',  ( -98.37445577226301907, -289.1458171220278928, -226.6842835789189223 ) ) ;
#90910=CARTESIAN_POINT ( 'NONE',  ( 3.296293995157008716, -276.1289521222244616, -208.8244452752689710 ) ) ;
#90911=CARTESIAN_POINT ( 'NONE',  ( 38.29064913625064293, -283.1145278293249703, -281.2401821678823239 ) ) ;
#90912=CARTESIAN_POINT ( 'NONE',  ( -45.91712290401081731, -295.9640262681513150, -195.4954454363450509 ) ) ;
#90913=CARTESIAN_POINT ( 'NONE',  ( -95.11644008230761926, -283.9236814554523107, -315.0030360031106511 ) ) ;
#90914=CARTESIAN_POINT ( 'NONE',  ( 19.44203619691334595, -276.3193363431988132, -223.5531890834425042 ) ) ;
#90915=CARTESIAN_POINT ( 'NONE',  ( 33.74585797779515417, -276.5833196329759289, -287.7101884586494975 ) ) ;
#90916=CARTESIAN_POINT ( 'NONE',  ( 35.39151566224521872, -285.8940188409931693, -290.8827277049616669 ) ) ;
#90917=CARTESIAN_POINT ( 'NONE',  ( -49.73721027179915666, -285.2102801604158344, -344.3821793724244458 ) ) ;
#90918=CARTESIAN_POINT ( 'NONE',  ( -110.6503002674750462, -271.5085867383893969, -267.6120100036642953 ) ) ;
#90920=CARTESIAN_POINT ( 'NONE',  ( 202.9738562182569694, 295.9636489450776367, -54.00000000004089173 ) ) ;
#90921=CARTESIAN_POINT ( 'NONE',  ( 39.22636708985139364, -293.2775039075388577, -261.7280272684386659 ) ) ;
#90922=CARTESIAN_POINT ( 'NONE',  ( -86.83518275965906241, -287.3399921341148229, -214.4149863381441889 ) ) ;
#90924=CARTESIAN_POINT ( 'NONE',  ( -99.86837403722181250, -282.6952119285918457, -220.4570493818173702 ) ) ;
#90925=CARTESIAN_POINT ( 'NONE',  ( -65.04641470917056267, -276.6020875286535556, -342.0874201227497338 ) ) ;
#90926=CARTESIAN_POINT ( 'NONE',  ( -84.68376105807472243, -288.0916404625320411, -330.1374955571340593 ) ) ;
#90928=CARTESIAN_POINT ( 'NONE',  ( 3.793132658930512324, -284.0078407313470734, -331.5672188670558853 ) ) ;
#90929=CARTESIAN_POINT ( 'NONE',  ( -37.79375931541365219, -278.8179959488529676, -344.3857002797081464 ) ) ;
#90930=CARTESIAN_POINT ( 'NONE',  ( -85.71522420497031192, -285.1321412110997358, -329.5101539820667540 ) ) ;
#90931=CARTESIAN_POINT ( 'NONE',  ( -42.97864262341066421, -281.9196614872113287, -343.5917704835240443 ) ) ;
#90932=CARTESIAN_POINT ( 'NONE',  ( -35.64233728854296146, -282.0736016031649456, -195.3676253642103688 ) ) ;
#90933=CARTESIAN_POINT ( 'NONE',  ( 13.96289506352593968, -274.9150602436251347, -212.8717651666284496 ) ) ;
#90934=CARTESIAN_POINT ( 'NONE',  ( -42.80828766433214838, -276.9526666038566987, -347.1668236639632710 ) ) ;
#90935=CARTESIAN_POINT ( 'NONE',  ( -20.49904834449667135, -296.7544872381379832, -342.9238354863966265 ) ) ;
#90939=CARTESIAN_POINT ( 'NONE',  ( -83.45253666998696929, -293.8158712047854806, -330.5446349255972223 ) ) ;
#90940=CARTESIAN_POINT ( 'NONE',  ( 23.84846012060114617, -274.5070845725301183, -230.4392852291380791 ) ) ;
#90941=CARTESIAN_POINT ( 'NONE',  ( -105.2640068955297323, -274.2177937244799182, -234.8265337162724222 ) ) ;
#90942=CARTESIAN_POINT ( 'NONE',  ( 25.80374816565178264, -288.7876104632247234, -231.7524871848097519 ) ) ;
#90943=CARTESIAN_POINT ( 'NONE',  ( -88.12940577804570808, -297.2675718264882789, -327.3820825954441034 ) ) ;
#90944=CARTESIAN_POINT ( 'NONE',  ( -111.2050540018490210, -297.5015775282732307, -290.6641639078940216 ) ) ;
#90945=CARTESIAN_POINT ( 'NONE',  ( -104.4792870326641179, -292.1153715076559934, -303.4152077143706379 ) ) ;
#90946=CARTESIAN_POINT ( 'NONE',  ( 10.46688989592492902, -278.7133933244763284, -212.7230083858162288 ) ) ;
#90947=CARTESIAN_POINT ( 'NONE',  ( -79.89773116671057096, -281.3916629014598243, -209.2849489982502007 ) ) ;
#90948=CARTESIAN_POINT ( 'NONE',  ( -96.76839655048529210, -294.0142223202572609, -315.2127163558214420 ) ) ;
#90949=CARTESIAN_POINT ( 'NONE',  ( -2.185909994324898520, -284.4522182847655358, -337.4757654372749585 ) ) ;
#90950=CARTESIAN_POINT ( 'NONE',  ( 27.93963876518999001, -286.0198847891174978, -236.8938997667564195 ) ) ;
#90951=CARTESIAN_POINT ( 'NONE',  ( 66.62391514549891269, 46.68937456676394504, -318.3441884561316328 ) ) ;
#90953=CARTESIAN_POINT ( 'NONE',  ( -99.62513603848654498, -284.7450927796080009, -232.1483733957276741 ) ) ;
#90955=CARTESIAN_POINT ( 'NONE',  ( 26.01744633488269542, -282.0585456217152114, -227.0583995882606985 ) ) ;
#90956=CARTESIAN_POINT ( 'NONE',  ( -96.30095538914154929, -273.4895104961962602, -227.1970191276514868 ) ) ;
#90957=CARTESIAN_POINT ( 'NONE',  ( -36.55402132116073233, -284.8567619757328089, -193.7492668471912509 ) ) ;
#90958=CARTESIAN_POINT ( 'NONE',  ( -25.44391599102797841, -281.1415039320959295, -194.5240363863448749 ) ) ;
#90959=CARTESIAN_POINT ( 'NONE',  ( 0.000000000000000000, 0.000000000000000000, 0.000000000000000000 ) ) ;
#90960=CARTESIAN_POINT ( 'NONE',  ( -73.45475546091442709, -281.1021299245235241, -203.1261023922344577 ) ) ;
#90961=CARTESIAN_POINT ( 'NONE',  ( -3.670690328810089831, -280.8176344348310067, -201.1222776717011129 ) ) ;
#90962=CARTESIAN_POINT ( 'NONE',  ( -37.30987171927208834, -289.5523547857346784, -200.3611179825600459 ) ) ;
#90963=CARTESIAN_POINT ( 'NONE',  ( -107.0744119028121446, -263.0355450277866680, -317.7147900177194515 ) ) ;
#90964=ORIENTED_EDGE ( 'NONE', *, *, #78083, .T. ) ;
#90965=CARTESIAN_POINT ( 'NONE',  ( -90.56350721584459507, -275.2960776685794144, -217.7543914547774477 ) ) ;
#90966=CARTESIAN_POINT ( 'NONE',  ( -56.85822679724589079, -169.0278465697174965, -364.1129473661134170 ) ) ;
#90967=CARTESIAN_POINT ( 'NONE',  ( 12.42068220339687201, -278.7695057721749663, -214.7234319704571419 ) ) ;
#90968=CARTESIAN_POINT ( 'NONE',  ( 36.43266382504649670, -295.0815434048254815, -252.1589961239934610 ) ) ;
#90969=CARTESIAN_POINT ( 'NONE',  ( -75.71862088245707412, -294.9273395214373750, -332.6383384075426761 ) ) ;
#90970=CARTESIAN_POINT ( 'NONE',  ( -13.87924978881762605, -291.8561594351979807, -197.0314506111629100 ) ) ;
#90972=CARTESIAN_POINT ( 'NONE',  ( -113.7772916893482460, -295.1007373478690852, -272.4355454230632745 ) ) ;
#90973=CARTESIAN_POINT ( 'NONE',  ( 34.78212824373949985, -285.7479476038117241, -254.7216231532430868 ) ) ;
#90974=CARTESIAN_POINT ( 'NONE',  ( 28.26054437331280411, -295.8792769279868935, -305.2159700821398474 ) ) ;
#90975=CARTESIAN_POINT ( 'NONE',  ( -96.30746453854132483, -285.2561239612773534, -314.2277580023124415 ) ) ;
#90977=CARTESIAN_POINT ( 'NONE',  ( 36.14793964560384865, -294.7747314882244041, -292.7244531363716646 ) ) ;
#90978=CARTESIAN_POINT ( 'NONE',  ( -37.53439365007844231, -283.5470123371905515, -343.4348423231849097 ) ) ;
#90979=CARTESIAN_POINT ( 'NONE',  ( -101.3052182973872135, -294.7888971317916571, -312.6077246920299899 ) ) ;
#90980=CARTESIAN_POINT ( 'NONE',  ( -108.2221289034982448, -291.7331115021885921, -240.6942402119126996 ) ) ;
#90981=CARTESIAN_POINT ( 'NONE',  ( -110.3744728098186272, -291.3512578876907924, -245.9922651095259312 ) ) ;
#90982=CARTESIAN_POINT ( 'NONE',  ( 27.03146753365539467, -288.1893873390139902, -304.8939219615119214 ) ) ;
#90985=CARTESIAN_POINT ( 'NONE',  ( -73.98780908681760593, -297.3936101085948280, -336.7325192630561332 ) ) ;
#90986=CARTESIAN_POINT ( 'NONE',  ( -27.03467378457320791, -272.9752015756983496, -194.4016130329067664 ) ) ;
#90987=CARTESIAN_POINT ( 'NONE',  ( -46.47395240873320432, -278.9923007490727969, -197.6461717106695630 ) ) ;
#90989=CARTESIAN_POINT ( 'NONE',  ( 26.88264667651773365, -274.5022752184702313, -227.9965079793375935 ) ) ;
#90990=CARTESIAN_POINT ( 'NONE',  ( -60.71765597359786426, -296.2233062917712232, -200.4195762110577448 ) ) ;
#90991=CARTESIAN_POINT ( 'NONE',  ( -5.729471905000831811, -278.4924110004315025, -337.5430645637092084 ) ) ;
#90992=CARTESIAN_POINT ( 'NONE',  ( -36.70202390154909011, -272.1998557082716843, -196.1160446736603546 ) ) ;
#90994=CARTESIAN_POINT ( 'NONE',  ( -84.72279142167131738, -296.9270242044190127, -326.4828334562519672 ) ) ;
#90995=CARTESIAN_POINT ( 'NONE',  ( -44.61337079273804562, -299.0377937805861848, -197.3629462935431889 ) ) ;
#90997=CARTESIAN_POINT ( 'NONE',  ( -51.67037220917357132, -299.4720675092139572, -195.4666458739050938 ) ) ;
#90999=CARTESIAN_POINT ( 'NONE',  ( -112.5377879941094932, -270.6443013071351515, -264.7236331678293482 ) ) ;
#91000=CARTESIAN_POINT ( 'NONE',  ( 8.906924158677348657, -293.3572351563867073, -213.6831234149605336 ) ) ;
#91001=CARTESIAN_POINT ( 'NONE',  ( -110.8961156397808736, -289.0803073707435260, -273.9194953613602479 ) ) ;
#91003=CARTESIAN_POINT ( 'NONE',  ( 37.88389657842101599, -275.8416498948889739, -254.1546182187037743 ) ) ;
#91004=CARTESIAN_POINT ( 'NONE',  ( 8.941184956592957533, -298.9805435559529201, -197.3372685744649004 ) ) ;
#91006=CARTESIAN_POINT ( 'NONE',  ( -76.65637301785764635, -281.5090867736279847, -206.0141283328111399 ) ) ;
#91007=CARTESIAN_POINT ( 'NONE',  ( -61.09457678357784260, -282.0388957169064952, -343.1426432866175560 ) ) ;
#91008=CARTESIAN_POINT ( 'NONE',  ( -28.62084665960789920, -276.2930346226852407, -346.8165820222291700 ) ) ;
#91009=CARTESIAN_POINT ( 'NONE',  ( -108.1824613252785241, -283.9901089479374718, -252.0803007027579383 ) ) ;
#91010=CARTESIAN_POINT ( 'NONE',  ( 36.61701703255067741, -279.7248558625624923, -283.8539762258984638 ) ) ;
#91012=CARTESIAN_POINT ( 'NONE',  ( -21.79196610406816603, -272.8300934221427951, -198.4335107151910904 ) ) ;
#91013=CARTESIAN_POINT ( 'NONE',  ( -43.25950329511469050, -279.1269158913100341, -345.1779740246709025 ) ) ;
#91016=CARTESIAN_POINT ( 'NONE',  ( -43.18911350981500163, -296.2192791470083080, -194.5472608965895347 ) ) ;
#91017=CARTESIAN_POINT ( 'NONE',  ( -45.42649278897774678, -279.1543904682803827, -345.1435258453242341 ) ) ;
#91018=CARTESIAN_POINT ( 'NONE',  ( -110.9623265619114960, -286.6890812506171642, -253.3517803642619697 ) ) ;
#91021=CARTESIAN_POINT ( 'NONE',  ( 35.27335428891451841, -285.7936672454010250, -289.1747137788573241 ) ) ;
#91023=CARTESIAN_POINT ( 'NONE',  ( -63.72598563317177423, -294.1987284430902037, -338.9058479885759994 ) ) ;
#91024=CARTESIAN_POINT ( 'NONE',  ( -20.87806073709151278, -286.9781783829336632, -342.7476778913273279 ) ) ;
#91025=CARTESIAN_POINT ( 'NONE',  ( 5.045406874201050940, -57.93311274753654061, -355.0152878038887820 ) ) ;
#91026=CARTESIAN_POINT ( 'NONE',  ( -101.9006828987354396, -294.0403003511833617, -308.6359176066416126 ) ) ;
#91027=CARTESIAN_POINT ( 'NONE',  ( 19.78071763164805930, -285.3397938032260299, -219.6892490331134127 ) ) ;
#91028=CARTESIAN_POINT ( 'NONE',  ( 36.31709171146466275, -283.0927441229456463, -265.7979175481778498 ) ) ;
#91029=CARTESIAN_POINT ( 'NONE',  ( 34.64182307317286558, -280.1045315314523236, -294.8626598633476306 ) ) ;
#91030=CARTESIAN_POINT ( 'NONE',  ( -42.66391403310464625, -289.1210224538163516, -343.2174499769024578 ) ) ;
#91031=CARTESIAN_POINT ( 'NONE',  ( -19.40839153056193922, -281.7125310320872700, -198.9377478122382001 ) ) ;
#91032=CARTESIAN_POINT ( 'NONE',  ( 31.21804926254937129, -282.0133906499681871, -244.6783577494234976 ) ) ;
#91033=CARTESIAN_POINT ( 'NONE',  ( 24.18720744861784056, -288.9434811833316417, -226.8348540555814736 ) ) ;
#91035=CARTESIAN_POINT ( 'NONE',  ( -111.0371254260475951, -272.8343313104732033, -247.8632948686687598 ) ) ;
#91036=CARTESIAN_POINT ( 'NONE',  ( -89.79945792042572350, -291.7768664939889618, -323.4650768636202542 ) ) ;
#91038=CARTESIAN_POINT ( 'NONE',  ( 25.18497378105907814, -289.4090924074130839, -220.4570493818173702 ) ) ;
#91040=CARTESIAN_POINT ( 'NONE',  ( -2.344454827926801599, -274.5899576281215673, -336.8834544615656910 ) ) ;
#91042=CARTESIAN_POINT ( 'NONE',  ( -66.63592358114750880, -293.8293853576281549, -340.7192490205051740 ) ) ;
#91043=CARTESIAN_POINT ( 'NONE',  ( -41.86589471663139506, -297.5012553282984413, -197.4397897920632943 ) ) ;
#91044=CARTESIAN_POINT ( 'NONE',  ( 20.06566681875769476, -289.7193814246786019, -316.5682816580791723 ) ) ;
#91045=CARTESIAN_POINT ( 'NONE',  ( -23.85921338480430620, -284.6376923185221699, -343.1360900701230321 ) ) ;
#91046=CARTESIAN_POINT ( 'NONE',  ( -110.6718409995223880, -292.2488860229383931, -248.8832984209662413 ) ) ;
#91047=CARTESIAN_POINT ( 'NONE',  ( -108.3345838939889063, -291.5030512620212448, -298.8796860788661434 ) ) ;
#91048=CARTESIAN_POINT ( 'NONE',  ( -49.77756589736652160, -287.8938299337074795, -196.3463920217268708 ) ) ;
#91049=CARTESIAN_POINT ( 'NONE',  ( -91.05968924537954479, -279.4814748918863643, -215.1199673354214212 ) ) ;
#91050=CARTESIAN_POINT ( 'NONE',  ( -102.5936827914308367, -295.1383954749189797, -232.1595972374336441 ) ) ;
#91051=CARTESIAN_POINT ( 'NONE',  ( 21.60864494763040611, -282.0524715603884829, -319.8975371101256542 ) ) ;
#91052=CARTESIAN_POINT ( 'NONE',  ( 31.43114174712345488, -277.7823219462227939, -298.4472752451638939 ) ) ;
#91053=CARTESIAN_POINT ( 'NONE',  ( -109.1418805571601069, -281.0519495502701943, -270.3937649182068412 ) ) ;
#91054=CARTESIAN_POINT ( 'NONE',  ( -34.36374767811492603, -275.1546732049775414, -346.0673745386463338 ) ) ;
#91057=CARTESIAN_POINT ( 'NONE',  ( 33.51680014956395581, -280.8244020716071532, -252.5040533427466585 ) ) ;
#91059=CARTESIAN_POINT ( 'NONE',  ( -100.1311941326400756, -279.1741332383115832, -314.2415026836567904 ) ) ;
#91060=CARTESIAN_POINT ( 'NONE',  ( -100.7952176068186390, -284.1834553710351656, -227.0645613887585057 ) ) ;
#91061=CARTESIAN_POINT ( 'NONE',  ( 28.37615571674690429, -294.8556181682639021, -236.3150105082035282 ) ) ;
#91062=CARTESIAN_POINT ( 'NONE',  ( 22.98685494044593369, -276.5242338031296754, -223.7898501736800085 ) ) ;
#91065=CARTESIAN_POINT ( 'NONE',  ( 35.25665166065600431, -276.5595717540737724, -246.0534453020507044 ) ) ;
#91067=CARTESIAN_POINT ( 'NONE',  ( 15.59641786974552602, -276.1100503125019259, -320.6259731733720173 ) ) ;
#91069=CARTESIAN_POINT ( 'NONE',  ( -105.3962054462466682, -298.9631972037566356, -239.1137557168918875 ) ) ;
#91070=CARTESIAN_POINT ( 'NONE',  ( -111.6973325211808827, -282.4375830948256976, -279.2514923850187074 ) ) ;
#91072=CARTESIAN_POINT ( 'NONE',  ( 38.30524771211417345, -293.0405107081077176, -256.1033631084205808 ) ) ;
#91073=CARTESIAN_POINT ( 'NONE',  ( -34.67420589349448790, -290.6192782274403612, -346.5144166086029145 ) ) ;
#91074=CARTESIAN_POINT ( 'NONE',  ( 33.61083317389190483, -292.2300831402139920, -251.9230027739928346 ) ) ;
#91076=CARTESIAN_POINT ( 'NONE',  ( -34.96045181805560276, -290.6562108069092574, -193.9744086591702512 ) ) ;
#91077=CARTESIAN_POINT ( 'NONE',  ( 32.65056747212670274, -292.9414288816075214, -249.3741081516795077 ) ) ;
#91079=CARTESIAN_POINT ( 'NONE',  ( -80.35582246825275377, -290.6993753544941796, -333.9176085439250983 ) ) ;
#91080=CARTESIAN_POINT ( 'NONE',  ( -98.01354234815093491, -279.4507005038909142, -229.6386417458874689 ) ) ;
#91081=CARTESIAN_POINT ( 'NONE',  ( -8.517028216829702458, -293.6040592334197186, -341.4851578888133190 ) ) ;
#91082=CARTESIAN_POINT ( 'NONE',  ( -69.75743829522463102, -286.2879006786095033, -200.6149081534760796 ) ) ;
#91083=CARTESIAN_POINT ( 'NONE',  ( 39.07011525867798696, -288.0074677189782051, -280.1162930545701784 ) ) ;
#91084=CARTESIAN_POINT ( 'NONE',  ( -56.32030779146403887, -283.6368112949385818, -340.8728186984362196 ) ) ;
#91085=CARTESIAN_POINT ( 'NONE',  ( -39.92122854846482483, -139.4860003333291445, -364.6914301237072777 ) ) ;
#91086=CARTESIAN_POINT ( 'NONE',  ( -79.00533470335423658, -207.5829368166174334, -355.8876102332309301 ) ) ;
#91087=CARTESIAN_POINT ( 'NONE',  ( 197.8626310074445200, 286.4972087208413427, -96.32890240008197225 ) ) ;
#91088=CARTESIAN_POINT ( 'NONE',  ( 23.19167250009359549, -274.1789077803798591, -229.2495619357918315 ) ) ;
#91089=CARTESIAN_POINT ( 'NONE',  ( -41.88943974837088291, -276.0310939175988665, -343.5416851109322920 ) ) ;
#91090=CARTESIAN_POINT ( 'NONE',  ( -114.1727638941521263, -295.9976242917600757, -275.3291459829642349 ) ) ;
#91091=CARTESIAN_POINT ( 'NONE',  ( -110.3257646060037445, -272.4678080593321852, -270.3600440800341289 ) ) ;
#91092=CARTESIAN_POINT ( 'NONE',  ( 31.40475345457193512, -274.6722214393019499, -304.0558796073630106 ) ) ;
#91093=CARTESIAN_POINT ( 'NONE',  ( -31.27873901767373610, -275.8898888938586538, -196.5837043736565022 ) ) ;
#91095=CARTESIAN_POINT ( 'NONE',  ( -92.95750875811738467, -274.3565290613117327, -217.5368902609039310 ) ) ;
#91097=CARTESIAN_POINT ( 'NONE',  ( 32.33038704787760764, -287.7526768366848273, -248.3240480478373229 ) ) ;
#91099=CARTESIAN_POINT ( 'NONE',  ( -61.53101358248718356, -296.1612786942654338, -343.3484580988664447 ) ) ;
#91100=CARTESIAN_POINT ( 'NONE',  ( -111.5310139230105619, -296.7889641599716697, -290.7442635200258110 ) ) ;
#91101=CARTESIAN_POINT ( 'NONE',  ( -72.12270919521363055, -295.6924067306260326, -334.5570150915633576 ) ) ;
#91103=( BOUNDED_SURFACE ( )  B_SPLINE_SURFACE ( 3, 2, ( 
 ( #49243, #78138, #76718, #71029, #51096, #36896, #93714, #7546, #71503, #51547, #43075, #86143, #79983, #14214, #86603, #87528, #65813, #923, #35969, #44451, #79537, #42588, #36430, #92784, #35516, #64889, #43982, #73358, #7098, #72429, #50649, #29339, #15581, #29803, #28869, #8005, #15120, #49700, #21772, #58684, #87077, #20831, #27953, #71979, #22675, #14676, #85684, #56843, #43532, #57757, #80436, #65346, #22226, #78596, #453, #35032, #13738, #58233, #63946, #6635, #72880, #64430, #93256, #28410, #57301, #21293, #50166, #79063, #15649, #30795, #81426, #22289, #50710, #51613, #80047, #15187, #36034, #8990, #80501, #65876, #44047, #51160, #72043, #8075, #88057, #72948, #985, #37869, #58295, #73423, #44519, #36963, #57819, #29866, #8533, #7159, #23214, #37412, #58751, #14738, #64951, #79597, #87593, #87138, #22739, #21835, #66321, #7605, #1436, #30321, #52550, #66774, #59211, #1905, #43593, #52094, #72489, #80978, #36493, #16121, #520, #43139, #44972 ),
 ( #73873, #59694, #88537, #23686, #52, #28933, #86670, #65410, #29404, #24137, #17979, #74331, #17045, #17523, #25537, #25999, #82373, #53959, #32184, #10857, #90838, #76210, #46373, #83289, #32661, #31264, #68172, #11339, #68644, #2386, #9455, #89451, #47292, #61088, #67254, #38341, #89929, #10392, #40191, #25085, #3776, #60151, #82826, #69110, #88990, #24609, #4235, #62003, #39257, #3293, #53015, #75733, #90382, #39720, #9932, #18435, #45911, #75273, #81892, #74817, #60613, #54418, #38806, #67710, #33115, #2840, #46831, #54884, #16575, #31722, #45430, #53497, #34530, #27424, #40651, #70987, #20789, #26486, #48713, #48241, #34989, #85179, #18919, #91324, #11800, #56314, #71458, #28367, #62967, #55376, #92267, #26952, #55841, #76673, #49661, #20329, #12766, #84696, #91801, #47773, #77617, #63906, #19843, #41608, #78556, #5191, #49199, #78094, #70530, #4698, #5655, #13236, #69570, #92741, #42072, #63438, #84228, #33575, #19375, #6119, #34065, #27912, #62484 ),
 ( #93215, #13693, #56799, #42545, #77143, #85641, #12274, #6594, #41117, #35471, #70049, #83763, #64389, #43490, #50120, #72386, #28831, #14632, #50604, #58190, #8881, #21729, #16014, #65301, #66214, #87032, #37308, #51978, #1794, #15078, #72835, #57258, #79496, #58641, #407, #80393, #15537, #7058, #86102, #44410, #21251, #35928, #7503, #79017, #14170, #43034, #881, #71936, #36388, #29295, #80867, #64846, #22184, #93673, #73317, #22633, #57714, #7961, #30212, #51052, #86559, #79940, #43938, #36856, #65772, #29761, #87483, #8429, #51505, #1330, #59103, #87944, #23095, #44866, #73769, #37761, #66666, #45321, #59579, #81783, #60505, #2734, #3188, #16933, #89340, #39607, #75168, #68063, #81320, #17872, #61448, #67141, #24495, #88882, #75627, #32072, #88430, #38228, #52446, #60969, #18331, #69003, #9826, #2275, #39151, #67606, #31614, #23579, #90279, #89820, #53376, #82262, #38699, #16467, #17415, #10750, #46264, #10281, #25430, #45794, #24981, #53855, #82720 ),
 ( #74224, #46724, #9343, #60044, #74705, #68531, #3668, #24030, #54308, #83183, #32556, #47187, #76099, #31158, #52906, #11232, #40086, #30679, #33464, #63325, #12647, #25889, #63792, #20209, #6006, #62857, #70422, #40544, #20679, #12163, #55266, #49087, #77032, #55730, #56685, #34881, #92621, #5071, #13581, #48600, #11693, #5548, #61896, #4591, #33953, #13126, #42433, #69929, #41492, #19732, #92156, #78445, #27792, #91690, #70875, #77985, #18812, #84582, #85532, #56199, #83648, #90730, #41006, #49550, #77500, #54771, #47669, #69459, #26842, #19271, #34418, #76570, #48129, #62367, #27313, #85058, #4134, #33005, #41962, #91210, #26378, #84121, #71823, #88659, #78899, #52671, #28714, #71343, #74455, #58878, #64273, #87724, #42909, #22875, #64729, #73549, #24265, #35815, #31387, #80633, #81552, #8658, #16700, #67380, #17177, #30448, #88192, #6473, #93556, #73997, #15789, #2038, #30928, #21136, #35351, #59818, #93102, #50006, #51740, #28257, #57145, #85986, #16245 ),
 ( #14046, #44648, #6942, #23808, #37990, #37536, #23352, #45555, #66447, #1565, #59340, #52219, #81102, #45095, #9114, #66898, #9588, #38476, #2510, #60277, #89114, #53140, #82020, #83408, #2960, #33235, #76801, #82499, #10979, #10515, #90962, #47427, #74946, #53629, #67835, #18560, #33706, #84349, #25205, #17647, #54540, #82948, #18102, #38926, #11927, #76337, #68772, #46955, #54078, #10056, #39849, #26126, #75857, #3901, #40776, #61218, #11463, #40314, #32778, #60735, #61666, #69229, #31846, #55022, #4358, #90498, #46498, #89575, #39384, #25658, #91458, #68299, #4823, #62131, #83892, #19043, #47899, #69694, #46041, #62618, #26609, #24747, #3420, #55500, #75401, #32315, #90052, #63091, #19498, #6720, #77268, #91919, #63560, #41243, #70185, #57833, #56920, #34187, #92387, #12894, #43155, #12397, #34648, #5319, #42667, #78674, #27074, #64027, #86221, #78214, #48365, #55960, #20452, #77743, #84814, #19964, #70646, #49319, #85303, #85759, #5774, #13353, #28485 ),
 ( #27547, #13815, #48837, #41732, #79146, #35593, #7174, #56440, #42194, #71107, #36048, #6239, #35108, #72057, #64966, #92868, #28031, #20909, #68, #49778, #71583, #64508, #28947, #93334, #57379, #21371, #50241, #14295, #73886, #1917, #79611, #29420, #73436, #65890, #36508, #38354, #15202, #7622, #88071, #72503, #22303, #44061, #23227, #22754, #51174, #52562, #81441, #52108, #80514, #9469, #87154, #80061, #1449, #65423, #87607, #72962, #80991, #30335, #14752, #16589, #9003, #88551, #51628, #59225, #58310, #67268, #1002, #8090, #86685, #23698, #36978, #43607, #29882, #58765, #15665, #44533, #8546, #2399, #37426, #45444, #66336, #30809, #16133, #66787, #74345, #31279, #44985, #37882, #21851, #59708, #50726, #535, #83304, #18450, #9947, #60164, #47309, #24150, #38819, #10407, #81906, #17059, #4715, #3793, #74834, #39271, #53511, #83779, #53029, #75287, #45924, #76224, #25552, #67725, #10871, #33130, #25100, #89003, #2854, #61104, #24626, #31736, #60627 ),
 ( #17537, #89943, #69124, #39734, #32675, #89465, #11355, #90854, #82389, #53973, #46388, #40208, #61562, #68188, #3309, #32198, #90394, #47789, #82841, #17994, #46847, #68657, #75748, #54432, #4251, #26018, #62019, #54901, #18934, #76691, #11816, #40668, #69586, #63452, #85195, #28383, #48731, #63921, #6134, #27439, #48258, #12785, #35005, #62502, #13708, #71003, #56332, #5209, #26502, #41135, #34544, #77635, #78111, #12290, #41626, #91817, #92759, #20805, #43049, #57274, #13251, #86117, #34082, #92283, #62985, #49674, #70068, #42560, #84713, #27926, #70546, #56815, #85657, #77160, #33594, #78570, #91340, #26969, #5669, #84244, #19394, #71953, #71477, #55860, #20344, #19861, #21266, #49215, #42086, #6609, #35489, #64403, #93230, #50137, #79036, #14188, #45341, #7072, #7980, #65319, #21746, #35944, #58207, #36874, #72853, #73335, #87052, #65789, #16033, #51524, #44429, #57730, #87963, #37779, #43506, #898, #426, #51999, #8446, #64862, #14650, #28846, #37325 ) ),
 .UNSPECIFIED., .T., .F., .T. ) 
 B_SPLINE_SURFACE_WITH_KNOTS ( ( 4, 3, 4 ),
 ( 3, 2, 2, 2, 2, 2, 2, 2, 2, 2, 2, 2, 2, 2, 2, 2, 2, 2, 2, 2, 2, 2, 2, 2, 2, 2, 2, 2, 2, 2, 2, 2, 2, 2, 2, 2, 2, 2, 2, 2, 2, 2, 2, 2, 2, 2, 2, 2, 2, 2, 2, 2, 2, 2, 2, 2, 2, 2, 2, 2, 2, 3 ),
 ( 0.000000000000000000, 0.5000000000000000000, 1.000000000000000000 ),
 ( -0.05855608392607185297, 0.000000000000000000, 0.01428571428571428527, 0.02857142857142857054, 0.04285714285714285754, 0.05714285714285714107, 0.07142857142857142461, 0.08571428571428571508, 0.1000000000000000056, 0.1142857142857142821, 0.1285714285714285587, 0.1428571428571428492, 0.1571428571428571397, 0.1714285714285714302, 0.1857142857142857206, 0.2000000000000000111, 0.2142857142857142738, 0.2285714285714285643, 0.2428571428571428548, 0.2571428571428571175, 0.2714285714285714080, 0.2857142857142856984, 0.2999999999999999889, 0.3142857142857142794, 0.3285714285714285698, 0.3428571428571428603, 0.3571428571428571508, 0.3714285714285714413, 0.3857142857142857317, 0.4000000000000000222, 0.4142857142857143127, 0.4285714285714285476, 0.4428571428571428381, 0.4571428571428571286, 0.4714285714285714191, 0.4857142857142857095, 0.5000000000000000000, 0.5142857142857142350, 0.5285714285714285809, 0.5428571428571428159, 0.5571428571428571619, 0.5714285714285713969, 0.5857142857142857428, 0.5999999999999999778, 0.6142857142857143238, 0.6285714285714285587, 0.6428571428571429047, 0.6571428571428571397, 0.6714285714285713746, 0.6857142857142857206, 0.6999999999999999556, 0.7142857142857143016, 0.7285714285714285365, 0.7428571428571428825, 0.7571428571428571175, 0.7714285714285714635, 0.7857142857142856984, 0.8000000000000000444, 0.8142857142857142794, 0.8285714285714286254, 0.8428571428571428603, 0.8500000000000000888 ),
 .UNSPECIFIED. ) 
 GEOMETRIC_REPRESENTATION_ITEM ( )  RATIONAL_B_SPLINE_SURFACE ( (
 ( 1.000000000000000000, 1.000000000000000000, 1.000000000000000000, 0.9749279121818236193, 1.000000000000000000, 0.9749279121818236193, 1.000000000000000000, 0.9749279121818236193, 1.000000000000000000, 0.9749279121818236193, 1.000000000000000000, 0.9749279121818236193, 1.000000000000000000, 0.9749279121818236193, 1.000000000000000000, 0.9749279121818236193, 1.000000000000000000, 0.9749279121818236193, 1.000000000000000000, 0.9749279121818236193, 1.000000000000000000, 0.9749279121818236193, 1.000000000000000000, 0.9749279121818236193, 1.000000000000000000, 0.9749279121818236193, 1.000000000000000000, 0.9749279121818236193, 1.000000000000000000, 0.9749279121818236193, 1.000000000000000000, 0.9749279121818236193, 1.000000000000000000, 0.9749279121818236193, 1.000000000000000000, 0.9749279121818236193, 1.000000000000000000, 0.9749279121818236193, 1.000000000000000000, 0.9749279121818236193, 1.000000000000000000, 0.9749279121818236193, 1.000000000000000000, 0.9749279121818236193, 1.000000000000000000, 0.9749279121818236193, 1.000000000000000000, 0.9749279121818236193, 1.000000000000000000, 0.9749279121818236193, 1.000000000000000000, 0.9749279121818236193, 1.000000000000000000, 0.9749279121818236193, 1.000000000000000000, 0.9749279121818236193, 1.000000000000000000, 0.9749279121818236193, 1.000000000000000000, 0.9749279121818236193, 1.000000000000000000, 0.9749279121818236193, 1.000000000000000000, 0.9749279121818236193, 1.000000000000000000, 0.9749279121818236193, 1.000000000000000000, 0.9749279121818236193, 1.000000000000000000, 0.9749279121818236193, 1.000000000000000000, 0.9749279121818236193, 1.000000000000000000, 0.9749279121818236193, 1.000000000000000000, 0.9749279121818236193, 1.000000000000000000, 0.9749279121818236193, 1.000000000000000000, 0.9749279121818236193, 1.000000000000000000, 0.9749279121818236193, 1.000000000000000000, 0.9749279121818236193, 1.000000000000000000, 0.9749279121818236193, 1.000000000000000000, 0.9749279121818236193, 1.000000000000000000, 0.9749279121818236193, 1.000000000000000000, 0.9749279121818236193, 1.000000000000000000, 0.9749279121818236193, 1.000000000000000000, 0.9749279121818236193, 1.000000000000000000, 0.9749279121818236193, 1.000000000000000000, 0.9749279121818236193, 1.000000000000000000, 0.9749279121818236193, 1.000000000000000000, 0.9749279121818236193, 1.000000000000000000, 0.9749279121818236193, 1.000000000000000000, 0.9749279121818236193, 1.000000000000000000, 0.9749279121818236193, 1.000000000000000000, 0.9749279121818236193, 1.000000000000000000, 0.9749279121818236193, 1.000000000000000000, 0.9749279121818236193, 1.000000000000000000, 0.9749279121818236193, 1.000000000000000000, 0.9749279121818236193, 1.000000000000000000, 0.9874639560909115321, 0.9874639560909117542),
 ( 0.3333333333333333703, 0.3333333333333333703, 0.3333333333333333703, 0.3249759707272745768, 0.3333333333333333703, 0.3249759707272745768, 0.3333333333333333703, 0.3249759707272745768, 0.3333333333333333703, 0.3249759707272745768, 0.3333333333333333703, 0.3249759707272745768, 0.3333333333333333703, 0.3249759707272745768, 0.3333333333333333703, 0.3249759707272745768, 0.3333333333333333703, 0.3249759707272745768, 0.3333333333333333703, 0.3249759707272745768, 0.3333333333333333703, 0.3249759707272745768, 0.3333333333333333703, 0.3249759707272745768, 0.3333333333333333703, 0.3249759707272745768, 0.3333333333333333703, 0.3249759707272745768, 0.3333333333333333703, 0.3249759707272745768, 0.3333333333333333703, 0.3249759707272745768, 0.3333333333333333703, 0.3249759707272745768, 0.3333333333333333703, 0.3249759707272745768, 0.3333333333333333703, 0.3249759707272745768, 0.3333333333333333703, 0.3249759707272745768, 0.3333333333333333703, 0.3249759707272745768, 0.3333333333333333703, 0.3249759707272745768, 0.3333333333333333703, 0.3249759707272745768, 0.3333333333333333703, 0.3249759707272745768, 0.3333333333333333703, 0.3249759707272745768, 0.3333333333333333703, 0.3249759707272745768, 0.3333333333333333703, 0.3249759707272745768, 0.3333333333333333703, 0.3249759707272745768, 0.3333333333333333703, 0.3249759707272745768, 0.3333333333333333703, 0.3249759707272745768, 0.3333333333333333703, 0.3249759707272745768, 0.3333333333333333703, 0.3249759707272745768, 0.3333333333333333703, 0.3249759707272745768, 0.3333333333333333703, 0.3249759707272745768, 0.3333333333333333703, 0.3249759707272745768, 0.3333333333333333703, 0.3249759707272745768, 0.3333333333333333703, 0.3249759707272745768, 0.3333333333333333703, 0.3249759707272745768, 0.3333333333333333703, 0.3249759707272745768, 0.3333333333333333703, 0.3249759707272745768, 0.3333333333333333703, 0.3249759707272745768, 0.3333333333333333703, 0.3249759707272745768, 0.3333333333333333703, 0.3249759707272745768, 0.3333333333333333703, 0.3249759707272745768, 0.3333333333333333703, 0.3249759707272745768, 0.3333333333333333703, 0.3249759707272745768, 0.3333333333333333703, 0.3249759707272745768, 0.3333333333333333703, 0.3249759707272745768, 0.3333333333333333703, 0.3249759707272745768, 0.3333333333333333703, 0.3249759707272745768, 0.3333333333333333703, 0.3249759707272745768, 0.3333333333333333703, 0.3249759707272745768, 0.3333333333333333703, 0.3249759707272745768, 0.3333333333333333703, 0.3249759707272745768, 0.3333333333333333703, 0.3249759707272745768, 0.3333333333333333703, 0.3249759707272745768, 0.3333333333333333703, 0.3249759707272745768, 0.3333333333333333703, 0.3249759707272745768, 0.3333333333333333703, 0.3249759707272745768, 0.3333333333333333703, 0.3249759707272745768, 0.3333333333333333703, 0.3291546520303039181, 0.3291546520303039736),
 ( 0.3333333333333333703, 0.3333333333333333703, 0.3333333333333333703, 0.3249759707272745768, 0.3333333333333333703, 0.3249759707272745768, 0.3333333333333333703, 0.3249759707272745768, 0.3333333333333333703, 0.3249759707272745768, 0.3333333333333333703, 0.3249759707272745768, 0.3333333333333333703, 0.3249759707272745768, 0.3333333333333333703, 0.3249759707272745768, 0.3333333333333333703, 0.3249759707272745768, 0.3333333333333333703, 0.3249759707272745768, 0.3333333333333333703, 0.3249759707272745768, 0.3333333333333333703, 0.3249759707272745768, 0.3333333333333333703, 0.3249759707272745768, 0.3333333333333333703, 0.3249759707272745768, 0.3333333333333333703, 0.3249759707272745768, 0.3333333333333333703, 0.3249759707272745768, 0.3333333333333333703, 0.3249759707272745768, 0.3333333333333333703, 0.3249759707272745768, 0.3333333333333333703, 0.3249759707272745768, 0.3333333333333333703, 0.3249759707272745768, 0.3333333333333333703, 0.3249759707272745768, 0.3333333333333333703, 0.3249759707272745768, 0.3333333333333333703, 0.3249759707272745768, 0.3333333333333333703, 0.3249759707272745768, 0.3333333333333333703, 0.3249759707272745768, 0.3333333333333333703, 0.3249759707272745768, 0.3333333333333333703, 0.3249759707272745768, 0.3333333333333333703, 0.3249759707272745768, 0.3333333333333333703, 0.3249759707272745768, 0.3333333333333333703, 0.3249759707272745768, 0.3333333333333333703, 0.3249759707272745768, 0.3333333333333333703, 0.3249759707272745768, 0.3333333333333333703, 0.3249759707272745768, 0.3333333333333333703, 0.3249759707272745768, 0.3333333333333333703, 0.3249759707272745768, 0.3333333333333333703, 0.3249759707272745768, 0.3333333333333333703, 0.3249759707272745768, 0.3333333333333333703, 0.3249759707272745768, 0.3333333333333333703, 0.3249759707272745768, 0.3333333333333333703, 0.3249759707272745768, 0.3333333333333333703, 0.3249759707272745768, 0.3333333333333333703, 0.3249759707272745768, 0.3333333333333333703, 0.3249759707272745768, 0.3333333333333333703, 0.3249759707272745768, 0.3333333333333333703, 0.3249759707272745768, 0.3333333333333333703, 0.3249759707272745768, 0.3333333333333333703, 0.3249759707272745768, 0.3333333333333333703, 0.3249759707272745768, 0.3333333333333333703, 0.3249759707272745768, 0.3333333333333333703, 0.3249759707272745768, 0.3333333333333333703, 0.3249759707272745768, 0.3333333333333333703, 0.3249759707272745768, 0.3333333333333333703, 0.3249759707272745768, 0.3333333333333333703, 0.3249759707272745768, 0.3333333333333333703, 0.3249759707272745768, 0.3333333333333333703, 0.3249759707272745768, 0.3333333333333333703, 0.3249759707272745768, 0.3333333333333333703, 0.3249759707272745768, 0.3333333333333333703, 0.3249759707272745768, 0.3333333333333333703, 0.3249759707272745768, 0.3333333333333333703, 0.3291546520303039181, 0.3291546520303039736),
 ( 1.000000000000000000, 1.000000000000000000, 1.000000000000000000, 0.9749279121818236193, 1.000000000000000000, 0.9749279121818236193, 1.000000000000000000, 0.9749279121818236193, 1.000000000000000000, 0.9749279121818236193, 1.000000000000000000, 0.9749279121818236193, 1.000000000000000000, 0.9749279121818236193, 1.000000000000000000, 0.9749279121818236193, 1.000000000000000000, 0.9749279121818236193, 1.000000000000000000, 0.9749279121818236193, 1.000000000000000000, 0.9749279121818236193, 1.000000000000000000, 0.9749279121818236193, 1.000000000000000000, 0.9749279121818236193, 1.000000000000000000, 0.9749279121818236193, 1.000000000000000000, 0.9749279121818236193, 1.000000000000000000, 0.9749279121818236193, 1.000000000000000000, 0.9749279121818236193, 1.000000000000000000, 0.9749279121818236193, 1.000000000000000000, 0.9749279121818236193, 1.000000000000000000, 0.9749279121818236193, 1.000000000000000000, 0.9749279121818236193, 1.000000000000000000, 0.9749279121818236193, 1.000000000000000000, 0.9749279121818236193, 1.000000000000000000, 0.9749279121818236193, 1.000000000000000000, 0.9749279121818236193, 1.000000000000000000, 0.9749279121818236193, 1.000000000000000000, 0.9749279121818236193, 1.000000000000000000, 0.9749279121818236193, 1.000000000000000000, 0.9749279121818236193, 1.000000000000000000, 0.9749279121818236193, 1.000000000000000000, 0.9749279121818236193, 1.000000000000000000, 0.9749279121818236193, 1.000000000000000000, 0.9749279121818236193, 1.000000000000000000, 0.9749279121818236193, 1.000000000000000000, 0.9749279121818236193, 1.000000000000000000, 0.9749279121818236193, 1.000000000000000000, 0.9749279121818236193, 1.000000000000000000, 0.9749279121818236193, 1.000000000000000000, 0.9749279121818236193, 1.000000000000000000, 0.9749279121818236193, 1.000000000000000000, 0.9749279121818236193, 1.000000000000000000, 0.9749279121818236193, 1.000000000000000000, 0.9749279121818236193, 1.000000000000000000, 0.9749279121818236193, 1.000000000000000000, 0.9749279121818236193, 1.000000000000000000, 0.9749279121818236193, 1.000000000000000000, 0.9749279121818236193, 1.000000000000000000, 0.9749279121818236193, 1.000000000000000000, 0.9749279121818236193, 1.000000000000000000, 0.9749279121818236193, 1.000000000000000000, 0.9749279121818236193, 1.000000000000000000, 0.9749279121818236193, 1.000000000000000000, 0.9749279121818236193, 1.000000000000000000, 0.9749279121818236193, 1.000000000000000000, 0.9749279121818236193, 1.000000000000000000, 0.9749279121818236193, 1.000000000000000000, 0.9749279121818236193, 1.000000000000000000, 0.9749279121818236193, 1.000000000000000000, 0.9749279121818236193, 1.000000000000000000, 0.9749279121818236193, 1.000000000000000000, 0.9874639560909115321, 0.9874639560909117542),
 ( 0.3333333333333333703, 0.3333333333333333703, 0.3333333333333333703, 0.3249759707272745768, 0.3333333333333333703, 0.3249759707272745768, 0.3333333333333333703, 0.3249759707272745768, 0.3333333333333333703, 0.3249759707272745768, 0.3333333333333333703, 0.3249759707272745768, 0.3333333333333333703, 0.3249759707272745768, 0.3333333333333333703, 0.3249759707272745768, 0.3333333333333333703, 0.3249759707272745768, 0.3333333333333333703, 0.3249759707272745768, 0.3333333333333333703, 0.3249759707272745768, 0.3333333333333333703, 0.3249759707272745768, 0.3333333333333333703, 0.3249759707272745768, 0.3333333333333333703, 0.3249759707272745768, 0.3333333333333333703, 0.3249759707272745768, 0.3333333333333333703, 0.3249759707272745768, 0.3333333333333333703, 0.3249759707272745768, 0.3333333333333333703, 0.3249759707272745768, 0.3333333333333333703, 0.3249759707272745768, 0.3333333333333333703, 0.3249759707272745768, 0.3333333333333333703, 0.3249759707272745768, 0.3333333333333333703, 0.3249759707272745768, 0.3333333333333333703, 0.3249759707272745768, 0.3333333333333333703, 0.3249759707272745768, 0.3333333333333333703, 0.3249759707272745768, 0.3333333333333333703, 0.3249759707272745768, 0.3333333333333333703, 0.3249759707272745768, 0.3333333333333333703, 0.3249759707272745768, 0.3333333333333333703, 0.3249759707272745768, 0.3333333333333333703, 0.3249759707272745768, 0.3333333333333333703, 0.3249759707272745768, 0.3333333333333333703, 0.3249759707272745768, 0.3333333333333333703, 0.3249759707272745768, 0.3333333333333333703, 0.3249759707272745768, 0.3333333333333333703, 0.3249759707272745768, 0.3333333333333333703, 0.3249759707272745768, 0.3333333333333333703, 0.3249759707272745768, 0.3333333333333333703, 0.3249759707272745768, 0.3333333333333333703, 0.3249759707272745768, 0.3333333333333333703, 0.3249759707272745768, 0.3333333333333333703, 0.3249759707272745768, 0.3333333333333333703, 0.3249759707272745768, 0.3333333333333333703, 0.3249759707272745768, 0.3333333333333333703, 0.3249759707272745768, 0.3333333333333333703, 0.3249759707272745768, 0.3333333333333333703, 0.3249759707272745768, 0.3333333333333333703, 0.3249759707272745768, 0.3333333333333333703, 0.3249759707272745768, 0.3333333333333333703, 0.3249759707272745768, 0.3333333333333333703, 0.3249759707272745768, 0.3333333333333333703, 0.3249759707272745768, 0.3333333333333333703, 0.3249759707272745768, 0.3333333333333333703, 0.3249759707272745768, 0.3333333333333333703, 0.3249759707272745768, 0.3333333333333333703, 0.3249759707272745768, 0.3333333333333333703, 0.3249759707272745768, 0.3333333333333333703, 0.3249759707272745768, 0.3333333333333333703, 0.3249759707272745768, 0.3333333333333333703, 0.3249759707272745768, 0.3333333333333333703, 0.3249759707272745768, 0.3333333333333333703, 0.3291546520303039181, 0.3291546520303039736),
 ( 0.3333333333333333703, 0.3333333333333333703, 0.3333333333333333703, 0.3249759707272745768, 0.3333333333333333703, 0.3249759707272745768, 0.3333333333333333703, 0.3249759707272745768, 0.3333333333333333703, 0.3249759707272745768, 0.3333333333333333703, 0.3249759707272745768, 0.3333333333333333703, 0.3249759707272745768, 0.3333333333333333703, 0.3249759707272745768, 0.3333333333333333703, 0.3249759707272745768, 0.3333333333333333703, 0.3249759707272745768, 0.3333333333333333703, 0.3249759707272745768, 0.3333333333333333703, 0.3249759707272745768, 0.3333333333333333703, 0.3249759707272745768, 0.3333333333333333703, 0.3249759707272745768, 0.3333333333333333703, 0.3249759707272745768, 0.3333333333333333703, 0.3249759707272745768, 0.3333333333333333703, 0.3249759707272745768, 0.3333333333333333703, 0.3249759707272745768, 0.3333333333333333703, 0.3249759707272745768, 0.3333333333333333703, 0.3249759707272745768, 0.3333333333333333703, 0.3249759707272745768, 0.3333333333333333703, 0.3249759707272745768, 0.3333333333333333703, 0.3249759707272745768, 0.3333333333333333703, 0.3249759707272745768, 0.3333333333333333703, 0.3249759707272745768, 0.3333333333333333703, 0.3249759707272745768, 0.3333333333333333703, 0.3249759707272745768, 0.3333333333333333703, 0.3249759707272745768, 0.3333333333333333703, 0.3249759707272745768, 0.3333333333333333703, 0.3249759707272745768, 0.3333333333333333703, 0.3249759707272745768, 0.3333333333333333703, 0.3249759707272745768, 0.3333333333333333703, 0.3249759707272745768, 0.3333333333333333703, 0.3249759707272745768, 0.3333333333333333703, 0.3249759707272745768, 0.3333333333333333703, 0.3249759707272745768, 0.3333333333333333703, 0.3249759707272745768, 0.3333333333333333703, 0.3249759707272745768, 0.3333333333333333703, 0.3249759707272745768, 0.3333333333333333703, 0.3249759707272745768, 0.3333333333333333703, 0.3249759707272745768, 0.3333333333333333703, 0.3249759707272745768, 0.3333333333333333703, 0.3249759707272745768, 0.3333333333333333703, 0.3249759707272745768, 0.3333333333333333703, 0.3249759707272745768, 0.3333333333333333703, 0.3249759707272745768, 0.3333333333333333703, 0.3249759707272745768, 0.3333333333333333703, 0.3249759707272745768, 0.3333333333333333703, 0.3249759707272745768, 0.3333333333333333703, 0.3249759707272745768, 0.3333333333333333703, 0.3249759707272745768, 0.3333333333333333703, 0.3249759707272745768, 0.3333333333333333703, 0.3249759707272745768, 0.3333333333333333703, 0.3249759707272745768, 0.3333333333333333703, 0.3249759707272745768, 0.3333333333333333703, 0.3249759707272745768, 0.3333333333333333703, 0.3249759707272745768, 0.3333333333333333703, 0.3249759707272745768, 0.3333333333333333703, 0.3249759707272745768, 0.3333333333333333703, 0.3249759707272745768, 0.3333333333333333703, 0.3291546520303039181, 0.3291546520303039736),
 ( 1.000000000000000000, 1.000000000000000000, 1.000000000000000000, 0.9749279121818236193, 1.000000000000000000, 0.9749279121818236193, 1.000000000000000000, 0.9749279121818236193, 1.000000000000000000, 0.9749279121818236193, 1.000000000000000000, 0.9749279121818236193, 1.000000000000000000, 0.9749279121818236193, 1.000000000000000000, 0.9749279121818236193, 1.000000000000000000, 0.9749279121818236193, 1.000000000000000000, 0.9749279121818236193, 1.000000000000000000, 0.9749279121818236193, 1.000000000000000000, 0.9749279121818236193, 1.000000000000000000, 0.9749279121818236193, 1.000000000000000000, 0.9749279121818236193, 1.000000000000000000, 0.9749279121818236193, 1.000000000000000000, 0.9749279121818236193, 1.000000000000000000, 0.9749279121818236193, 1.000000000000000000, 0.9749279121818236193, 1.000000000000000000, 0.9749279121818236193, 1.000000000000000000, 0.9749279121818236193, 1.000000000000000000, 0.9749279121818236193, 1.000000000000000000, 0.9749279121818236193, 1.000000000000000000, 0.9749279121818236193, 1.000000000000000000, 0.9749279121818236193, 1.000000000000000000, 0.9749279121818236193, 1.000000000000000000, 0.9749279121818236193, 1.000000000000000000, 0.9749279121818236193, 1.000000000000000000, 0.9749279121818236193, 1.000000000000000000, 0.9749279121818236193, 1.000000000000000000, 0.9749279121818236193, 1.000000000000000000, 0.9749279121818236193, 1.000000000000000000, 0.9749279121818236193, 1.000000000000000000, 0.9749279121818236193, 1.000000000000000000, 0.9749279121818236193, 1.000000000000000000, 0.9749279121818236193, 1.000000000000000000, 0.9749279121818236193, 1.000000000000000000, 0.9749279121818236193, 1.000000000000000000, 0.9749279121818236193, 1.000000000000000000, 0.9749279121818236193, 1.000000000000000000, 0.9749279121818236193, 1.000000000000000000, 0.9749279121818236193, 1.000000000000000000, 0.9749279121818236193, 1.000000000000000000, 0.9749279121818236193, 1.000000000000000000, 0.9749279121818236193, 1.000000000000000000, 0.9749279121818236193, 1.000000000000000000, 0.9749279121818236193, 1.000000000000000000, 0.9749279121818236193, 1.000000000000000000, 0.9749279121818236193, 1.000000000000000000, 0.9749279121818236193, 1.000000000000000000, 0.9749279121818236193, 1.000000000000000000, 0.9749279121818236193, 1.000000000000000000, 0.9749279121818236193, 1.000000000000000000, 0.9749279121818236193, 1.000000000000000000, 0.9749279121818236193, 1.000000000000000000, 0.9749279121818236193, 1.000000000000000000, 0.9749279121818236193, 1.000000000000000000, 0.9749279121818236193, 1.000000000000000000, 0.9749279121818236193, 1.000000000000000000, 0.9749279121818236193, 1.000000000000000000, 0.9749279121818236193, 1.000000000000000000, 0.9874639560909115321, 0.9874639560909117542) ) ) 
 REPRESENTATION_ITEM ( '' )  SURFACE ( )  );
#91104=CARTESIAN_POINT ( 'NONE',  ( 18.82351850331043863, -278.1715975867599582, -320.9253439018280005 ) ) ;
#91106=CARTESIAN_POINT ( 'NONE',  ( -40.99919221731766328, -279.5149707911952532, -193.4964550853976561 ) ) ;
#91107=CARTESIAN_POINT ( 'NONE',  ( 20.21480145023641839, -277.1303281130089431, -315.6655045440019194 ) ) ;
#91108=CARTESIAN_POINT ( 'NONE',  ( 7.659227149099407939, -278.2078693657250597, -331.6544610544016223 ) ) ;
#91109=CARTESIAN_POINT ( 'NONE',  ( -79.33105313509143741, -275.6355789438951547, -332.9963122945742384 ) ) ;
#91110=CARTESIAN_POINT ( 'NONE',  ( -14.05175544632568041, -274.8549589020640838, -201.1110860814869170 ) ) ;
#91111=CARTESIAN_POINT ( 'NONE',  ( -61.22139527606407938, -293.9429678346589299, -340.0221344507196477 ) ) ;
#91113=CARTESIAN_POINT ( 'NONE',  ( 30.66448207899649603, -281.5782029110057465, -234.2658066876924181 ) ) ;
#91114=CARTESIAN_POINT ( 'NONE',  ( -110.1681798653654880, -278.6433785491622643, -276.0809966728783706 ) ) ;
#91115=CARTESIAN_POINT ( 'NONE',  ( 16.32799796159937245, -286.9944393058921150, -324.9587260141474303 ) ) ;
#91116=CARTESIAN_POINT ( 'NONE',  ( -21.79489099465742186, -276.2515857259405720, -196.9901607077368340 ) ) ;
#91119=CARTESIAN_POINT ( 'NONE',  ( -48.09479457895627519, -288.3894816949112396, -342.7791843982212185 ) ) ;
#91120=CARTESIAN_POINT ( 'NONE',  ( -90.37385592451531124, -283.1274661494136353, -326.1198924788092199 ) ) ;
#91121=CARTESIAN_POINT ( 'NONE',  ( -0.7705315264256661356, -280.7991299456670617, -334.7080187723231006 ) ) ;
#91122=CARTESIAN_POINT ( 'NONE',  ( 26.98261595473158181, -279.6420769262680324, -234.6153871012163847 ) ) ;
#91123=CARTESIAN_POINT ( 'NONE',  ( -80.11715233710630457, -283.5483958948841519, -209.3751547080865691 ) ) ;
#91124=CARTESIAN_POINT ( 'NONE',  ( -49.77975540794616194, -287.8937990868191150, -196.3475945179768587 ) ) ;
#91125=CARTESIAN_POINT ( 'NONE',  ( -68.70682381515995019, -280.8354766992522400, -204.0033036554774526 ) ) ;
#91127=CIRCLE ( 'NONE', #88099, 3.491568894204821749 ) ;
#91128=CARTESIAN_POINT ( 'NONE',  ( -66.26823076813668933, -293.6736317085897667, -201.1638891686486375 ) ) ;
#91129=CARTESIAN_POINT ( 'NONE',  ( -71.14053061027676961, -275.7320125167084370, -338.4170734547194002 ) ) ;
#91131=CARTESIAN_POINT ( 'NONE',  ( -64.36311352750779236, -278.0656231866486792, -338.3393588691618561 ) ) ;
#91132=CARTESIAN_POINT ( 'NONE',  ( -110.4303697114122116, -286.3267434986474882, -287.9675886507163796 ) ) ;
#91135=CARTESIAN_POINT ( 'NONE',  ( 104.1717476309105166, -299.5541904835127980, -195.3611179825600175 ) ) ;
#91136=CARTESIAN_POINT ( 'NONE',  ( -111.1533240022837816, -292.2663411257876760, -286.5215135008785410 ) ) ;
#91138=CARTESIAN_POINT ( 'NONE',  ( -38.21988350492071618, -293.0630105629219315, -345.3685269068163848 ) ) ;
#91139=CARTESIAN_POINT ( 'NONE',  ( -30.88720699871515762, -285.3289064184366453, -193.7808977009793523 ) ) ;
#91141=CARTESIAN_POINT ( 'NONE',  ( 35.51155968610129321, -274.1101725387546253, -260.6840310026798306 ) ) ;
#91142=CARTESIAN_POINT ( 'NONE',  ( -41.12548022622988242, -293.2398284290188144, -344.5126089476709694 ) ) ;
#91145=CARTESIAN_POINT ( 'NONE',  ( -70.57807687372837790, -290.1017145325866977, -201.6730475722353049 ) ) ;
#91146=CARTESIAN_POINT ( 'NONE',  ( -41.38693288121886837, -287.6005376149668677, -196.6594299747017374 ) ) ;
#91147=CARTESIAN_POINT ( 'NONE',  ( 21.60467206546135088, -286.4441540502930366, -318.3325962722149711 ) ) ;
#91149=CARTESIAN_POINT ( 'NONE',  ( -101.5139699641699451, -286.4675323826448334, -234.2386648065198074 ) ) ;
#91151=CARTESIAN_POINT ( 'NONE',  ( 0.2428599936132283532, -287.3690090560045292, -207.5326206330393575 ) ) ;
#91152=CARTESIAN_POINT ( 'NONE',  ( 36.15142411509117437, -295.3186181277409332, -253.6550036725486734 ) ) ;
#91153=CARTESIAN_POINT ( 'NONE',  ( -39.93842410471280857, -275.1643568117752920, -345.8893103126946471 ) ) ;
#91154=CARTESIAN_POINT ( 'NONE',  ( 19.86433370714091851, -276.5849809431883273, -321.8902041055885093 ) ) ;
#91156=CARTESIAN_POINT ( 'NONE',  ( 25.31281544100516001, -291.0638748786709016, -228.0348577190633534 ) ) ;
#91157=CARTESIAN_POINT ( 'NONE',  ( -77.49251644047828336, -279.5295137937271761, -204.5961810932253115 ) ) ;
#91158=CARTESIAN_POINT ( 'NONE',  ( -69.19687180141157512, -297.4530941586672270, -337.8814147295076395 ) ) ;
#91160=DIRECTION ( 'NONE',  ( 0.000000000000000000, 0.000000000000000000, 1.000000000000000000 ) ) ;
#91161=CARTESIAN_POINT ( 'NONE',  ( -11.83523223400857205, -285.0761274482836143, -201.4360603221494159 ) ) ;
#91162=CARTESIAN_POINT ( 'NONE',  ( -81.57403355917152510, -275.8009975677020407, -329.9796231370935402 ) ) ;
#91163=CARTESIAN_POINT ( 'NONE',  ( 33.44863614909306904, -279.2294068253228261, -245.4322969748367882 ) ) ;
#91165=CARTESIAN_POINT ( 'NONE',  ( 25.58388106276237295, -273.4569774017685972, -227.1745515018921822 ) ) ;
#91166=CARTESIAN_POINT ( 'NONE',  ( -107.9208395050715552, -277.6496055655351824, -289.3999665096213789 ) ) ;
#91167=CARTESIAN_POINT ( 'NONE',  ( 4.223254074979974071, -296.0005677408698261, -331.2139103030986576 ) ) ;
#91169=CARTESIAN_POINT ( 'NONE',  ( -38.15278955346298062, -278.9625449387969525, -193.6745178159125658 ) ) ;
#91170=CARTESIAN_POINT ( 'NONE',  ( -34.27939665490124099, -295.9539623870759328, -343.5323605991071645 ) ) ;
#91171=CARTESIAN_POINT ( 'NONE',  ( -104.8265627010655834, -298.3373609539154927, -234.2057751478373007 ) ) ;
#91172=CARTESIAN_POINT ( 'NONE',  ( -92.74302058066339782, -297.0623615167057778, -222.8056558867747867 ) ) ;
#91173=CARTESIAN_POINT ( 'NONE',  ( -66.11723532431140882, -293.6757415129305286, -201.0870750876899820 ) ) ;
#91174=CARTESIAN_POINT ( 'NONE',  ( -100.9976888636195582, -285.2912086263243623, -226.9435482991604829 ) ) ;
#91175=CARTESIAN_POINT ( 'NONE',  ( 36.74267169341347739, -273.4892675108972071, -254.4311332663733936 ) ) ;
#91176=CARTESIAN_POINT ( 'NONE',  ( 30.36167868341750165, -287.8611994579429165, -307.1503073310834679 ) ) ;
#91177=CARTESIAN_POINT ( 'NONE',  ( -110.7542260487683166, -280.7063025978318365, -256.8537924575717852 ) ) ;
#91178=CARTESIAN_POINT ( 'NONE',  ( 35.19174914420086964, -286.7450961431770793, -280.5670182140430597 ) ) ;
#91179=CARTESIAN_POINT ( 'NONE',  ( -110.6169402856506565, -288.3466611573664977, -286.3529856975630423 ) ) ;
#91181=CARTESIAN_POINT ( 'NONE',  ( 134.9260051231060800, 178.6636279401649858, -236.0341445084446548 ) ) ;
#91182=CARTESIAN_POINT ( 'NONE',  ( -23.77989730216035724, -288.3819591849186850, -342.2046832395990918 ) ) ;
#91183=CARTESIAN_POINT ( 'NONE',  ( -61.14728354254373954, -284.2949582614295423, -343.3968618803212394 ) ) ;
#91184=CARTESIAN_POINT ( 'NONE',  ( -98.15449028097435757, -290.2381848154611816, -223.4930305982076959 ) ) ;
#91185=CARTESIAN_POINT ( 'NONE',  ( 38.83995597524599930, -283.1107051754440249, -267.0713769925428096 ) ) ;
#91187=CARTESIAN_POINT ( 'NONE',  ( -59.17751767948421815, -281.0904549733824069, -197.0365290405921428 ) ) ;
#91188=CARTESIAN_POINT ( 'NONE',  ( 28.97357045158723210, -280.9723223964496128, -239.7230077796126579 ) ) ;
#91189=CARTESIAN_POINT ( 'NONE',  ( 0.4398160855076280740, -276.5556580843460210, -205.5575686543582492 ) ) ;
#91190=CARTESIAN_POINT ( 'NONE',  ( -34.85464314124794782, -295.0217161261292063, -347.3209422257600636 ) ) ;
#91191=CARTESIAN_POINT ( 'NONE',  ( -98.08548462581161687, -289.1660821441731173, -226.8912489125631851 ) ) ;
#91192=CARTESIAN_POINT ( 'NONE',  ( 52.15744429099725465, -298.1187141199046664, -197.0689410925062361 ) ) ;
#91193=ORIENTED_EDGE ( 'NONE', *, *, #33593, .T. ) ;
#91195=CARTESIAN_POINT ( 'NONE',  ( -94.51261618817551380, -285.8088720643203828, -318.0350160593292230 ) ) ;
#91197=CARTESIAN_POINT ( 'NONE',  ( -70.66109363059125315, -296.5608803184114208, -339.4502423935154525 ) ) ;
#91198=CARTESIAN_POINT ( 'NONE',  ( 14.00217284268275186, -282.9598814247329415, -322.4679566670448594 ) ) ;
#91199=CARTESIAN_POINT ( 'NONE',  ( 24.17190392111125874, -275.2236974222782919, -316.2838436256404862 ) ) ;
#91200=CARTESIAN_POINT ( 'NONE',  ( -88.58773585299572062, -292.0066231195654041, -213.0273878685330260 ) ) ;
#91201=CARTESIAN_POINT ( 'NONE',  ( -33.76160766181091333, -284.2363424040913173, -194.6809460743868101 ) ) ;
#91202=CARTESIAN_POINT ( 'NONE',  ( 8.834851233142318350, -292.9990086904267059, -208.7034376754828884 ) ) ;
#91204=CARTESIAN_POINT ( 'NONE',  ( -94.11804822104657831, -290.2361271288630746, -316.2798917477898044 ) ) ;
#91205=CARTESIAN_POINT ( 'NONE',  ( 115.2448031289451222, -299.5541904835127980, -198.2496582146980302 ) ) ;
#91207=DIRECTION ( 'NONE',  ( 1.000000000000000000, 0.000000000000000000, 0.000000000000000000 ) ) ;
#91208=CARTESIAN_POINT ( 'NONE',  ( -82.19941185436130127, -219.0997270613688670, -349.0470628824017467 ) ) ;
#91209=CARTESIAN_POINT ( 'NONE',  ( -83.44872848485381667, -285.1911182727992013, -331.2292047662632513 ) ) ;
#91210=CARTESIAN_POINT ( 'NONE',  ( 39.58706461736021254, -279.0523547857347921, -270.3937649182068981 ) ) ;
#91212=CARTESIAN_POINT ( 'NONE',  ( 35.00641068001061029, -280.6278915892891632, -282.1923028971748408 ) ) ;
#91213=CARTESIAN_POINT ( 'NONE',  ( -28.60765223002002600, -276.6111153869907184, -346.8964454929711110 ) ) ;
#91214=CARTESIAN_POINT ( 'NONE',  ( -109.7528847541661889, -280.7961214315325833, -251.4255698042724418 ) ) ;
#91215=CARTESIAN_POINT ( 'NONE',  ( -37.45856812746255571, -140.9159241237307185, -362.6039797469185260 ) ) ;
#91216=CARTESIAN_POINT ( 'NONE',  ( -1.396452039911038723, -279.0940891009174152, -202.9330419764321221 ) ) ;
#91218=CARTESIAN_POINT ( 'NONE',  ( -63.10747744129525927, -283.7351743835561138, -200.2490867062971915 ) ) ;
#91219=CARTESIAN_POINT ( 'NONE',  ( -37.62665763008747888, -299.8087642997211901, -194.3749822932419704 ) ) ;
#91221=CARTESIAN_POINT ( 'NONE',  ( 18.88446801193410352, -294.7056354384393444, -317.0152331080279282 ) ) ;
#91223=CARTESIAN_POINT ( 'NONE',  ( -105.1516594518534617, -289.6161362530509109, -241.8905698363981287 ) ) ;
#91224=CARTESIAN_POINT ( 'NONE',  ( -5.319649073906242975, -277.2931421010299573, -340.2746433786214197 ) ) ;
#91225=CARTESIAN_POINT ( 'NONE',  ( 33.50918050270857407, -275.3201304803966991, -252.7783788944213939 ) ) ;
#91226=CARTESIAN_POINT ( 'NONE',  ( 24.23990536485205283, -273.8623176863985123, -224.6533683608712124 ) ) ;
#91228=CARTESIAN_POINT ( 'NONE',  ( -112.3407595013127604, -270.5879613108983222, -267.5593803803137689 ) ) ;
#91233=CARTESIAN_POINT ( 'NONE',  ( 1.275780383236181370, -283.6032046678731717, -332.7334504865265785 ) ) ;
#91234=CARTESIAN_POINT ( 'NONE',  ( 15.07100037025026040, -284.0848382429485355, -325.3782320343473202 ) ) ;
#91235=CARTESIAN_POINT ( 'NONE',  ( -95.20220198837948544, -283.2723736632433997, -315.0587855295223676 ) ) ;
#91236=CARTESIAN_POINT ( 'NONE',  ( 33.63499765952607845, -273.6854549047521914, -249.9607960373914750 ) ) ;
#91237=CARTESIAN_POINT ( 'NONE',  ( 22.30758168845396838, -282.8029982556293476, -226.1489109688006636 ) ) ;
#91238=CARTESIAN_POINT ( 'NONE',  ( -99.77267198196132370, -276.4953160061438098, -309.6110597349018576 ) ) ;
#91240=CARTESIAN_POINT ( 'NONE',  ( 17.50772282984454620, -275.9390178205849224, -221.6467668302588265 ) ) ;
#91242=CARTESIAN_POINT ( 'NONE',  ( -22.60718213729673565, -281.0388419842026906, -194.8944267758628541 ) ) ;
#91246=CARTESIAN_POINT ( 'NONE',  ( -29.61287910174063143, -288.0094571674408144, -194.9915564524682168 ) ) ;
#91247=CARTESIAN_POINT ( 'NONE',  ( -68.59558629629512438, -294.6708202636175429, -336.5246824996507939 ) ) ;
#91248=CARTESIAN_POINT ( 'NONE',  ( -114.1498885402841807, -289.8541943165051862, -274.0779686834404743 ) ) ;
#91249=CARTESIAN_POINT ( 'NONE',  ( 19.45358290260161738, -285.1274609166684399, -222.8832804056557393 ) ) ;
#91250=CARTESIAN_POINT ( 'NONE',  ( 9.418773466919910575, -285.2845214201378781, -213.5382966463484422 ) ) ;
#91251=CARTESIAN_POINT ( 'NONE',  ( -99.13335567182939201, -289.3504158651628586, -229.5278475491807626 ) ) ;
#91252=CARTESIAN_POINT ( 'NONE',  ( -106.9135861263490312, -286.0680764986466897, -246.8163411235290141 ) ) ;
#91253=CARTESIAN_POINT ( 'NONE',  ( 0.02781816129643214022, -274.5550432056894010, -335.4470851720672613 ) ) ;
#91254=CARTESIAN_POINT ( 'NONE',  ( 13.72600977953973533, -285.1532728594528976, -213.7347662021486201 ) ) ;
#91255=CARTESIAN_POINT ( 'NONE',  ( -96.66802440740052305, -299.1813919990765385, -224.4558752512333228 ) ) ;
#91256=CARTESIAN_POINT ( 'NONE',  ( 27.13926965407637937, -285.0347991584364991, -231.6312483817269197 ) ) ;
#91257=CARTESIAN_POINT ( 'NONE',  ( 18.13494964482363514, -281.8144718828905297, -222.5323560032991850 ) ) ;
#91258=CARTESIAN_POINT ( 'NONE',  ( -81.74855100402548658, -291.6555331162216476, -331.0081296070798089 ) ) ;
#91261=CARTESIAN_POINT ( 'NONE',  ( -50.19799470182257295, -297.1350241498703895, -344.8722944920820623 ) ) ;
#91262=CARTESIAN_POINT ( 'NONE',  ( -77.88208727294285438, -277.5077983827608819, -207.2002697336634185 ) ) ;
#91263=CARTESIAN_POINT ( 'NONE',  ( -3.383483752952189949, -291.6862626266616871, -201.4191233759826218 ) ) ;
#91264=CARTESIAN_POINT ( 'NONE',  ( -108.3783306260521471, -294.6904311970313870, -290.3670556954279505 ) ) ;
#91265=CARTESIAN_POINT ( 'NONE',  ( 8.085731424016778135, -281.1012431243286755, -328.1979967438466588 ) ) ;
#91266=CARTESIAN_POINT ( 'NONE',  ( -13.58314515275353784, -272.4428463835358798, -199.8143585816483210 ) ) ;
#91267=CARTESIAN_POINT ( 'NONE',  ( 25.25921100355509452, -294.3389911268475316, -231.7629899049199480 ) ) ;
#91268=CARTESIAN_POINT ( 'NONE',  ( -4.771743288812468897, -291.1233781216987495, -337.9199732462171255 ) ) ;
#91269=CARTESIAN_POINT ( 'NONE',  ( -97.73767100012669573, -294.4038934749632972, -316.9983826705367278 ) ) ;
#91270=CARTESIAN_POINT ( 'NONE',  ( -8.789871987137727771, -292.9236992624399818, -340.8353620211534007 ) ) ;
#91271=CARTESIAN_POINT ( 'NONE',  ( -110.5609595067740543, -292.0738732060030998, -262.9912487543835482 ) ) ;
#91273=CARTESIAN_POINT ( 'NONE',  ( -67.87788778166178361, -292.4436131836936283, -203.8631964398795162 ) ) ;
#91275=CARTESIAN_POINT ( 'NONE',  ( 1.230095228631854498, -280.5598161610066086, -335.0961425483314997 ) ) ;
#91276=CARTESIAN_POINT ( 'NONE',  ( -17.43259608145457307, -292.3161704390975615, -200.0758581772058449 ) ) ;
#91278=CARTESIAN_POINT ( 'NONE',  ( 17.22311194634449549, -280.8043158201616620, -215.9569753895094095 ) ) ;
#91279=CARTESIAN_POINT ( 'NONE',  ( -86.09225791230193181, -283.3738707646173225, -329.9356713351689336 ) ) ;
#91280=CARTESIAN_POINT ( 'NONE',  ( 11.28777492635730084, -286.3767784430328334, -327.3084558805859956 ) ) ;
#91281=CARTESIAN_POINT ( 'NONE',  ( -85.68378825524501963, -281.8692161328968382, -326.6985655031110696 ) ) ;
#91282=CARTESIAN_POINT ( 'NONE',  ( 24.04559783597816747, -279.4242473727307470, -225.0366499457509804 ) ) ;
#91284=CARTESIAN_POINT ( 'NONE',  ( 28.44050858424596839, -285.9551399711476734, -230.8354079063705626 ) ) ;
#91286=CARTESIAN_POINT ( 'NONE',  ( 35.11364362255328331, -295.3352736961820142, -284.3847972003716222 ) ) ;
#91287=CARTESIAN_POINT ( 'NONE',  ( -38.51754974594984304, -278.4918911310675185, -346.7628435698167095 ) ) ;
#91288=CARTESIAN_POINT ( 'NONE',  ( -80.83537442462778699, -277.3278865263428656, -329.0159369053936302 ) ) ;
#91289=CARTESIAN_POINT ( 'NONE',  ( -100.0322822802275624, -291.3109982988033266, -225.6521601112227984 ) ) ;
#91291=CARTESIAN_POINT ( 'NONE',  ( 10.56045666592079257, -280.4767086457568439, -328.8642206116721809 ) ) ;
#91294=CARTESIAN_POINT ( 'NONE',  ( 16.92056002333560727, -291.9077598748362448, -221.1032366057138461 ) ) ;
#91295=CARTESIAN_POINT ( 'NONE',  ( -99.08921189694146392, -295.1292966939730036, -227.7680830393643134 ) ) ;
#91298=CARTESIAN_POINT ( 'NONE',  ( 35.35722735411813744, -292.9575275240945871, -262.6016047728442686 ) ) ;
#91299=DIRECTION ( 'NONE',  ( 1.000000000000000000, 0.000000000000000000, 0.000000000000000000 ) ) ;
#91300=CARTESIAN_POINT ( 'NONE',  ( -92.08974858914540107, -287.4094976428775112, -313.9805196606274080 ) ) ;
#91301=CARTESIAN_POINT ( 'NONE',  ( 30.54179879548563292, -297.9412943616089251, -193.6069287863579689 ) ) ;
#91302=CARTESIAN_POINT ( 'NONE',  ( -2.929649398343377786, -278.6415350863802018, -202.8476154217746341 ) ) ;
#91303=CARTESIAN_POINT ( 'NONE',  ( -57.64131366847546190, -287.1106933631196512, -196.5414649848554802 ) ) ;
#91304=CARTESIAN_POINT ( 'NONE',  ( -45.36455647170634364, -288.9899505576246383, -342.9189141218286068 ) ) ;
#91305=CARTESIAN_POINT ( 'NONE',  ( -111.0856700441927813, -280.0683763114077465, -270.6600037201490636 ) ) ;
#91306=CARTESIAN_POINT ( 'NONE',  ( -110.2027499684331389, -294.3629977138155027, -286.5819139941789899 ) ) ;
#91307=CARTESIAN_POINT ( 'NONE',  ( -93.84163265591229219, -297.6418946340604634, -318.1900699764167371 ) ) ;
#91309=CARTESIAN_POINT ( 'NONE',  ( -85.37663542332029465, -276.5281358890228489, -325.9241800736950836 ) ) ;
#91311=CARTESIAN_POINT ( 'NONE',  ( -108.0766608621983238, -272.7745362790577133, -239.8031790565791823 ) ) ;
#91312=CARTESIAN_POINT ( 'NONE',  ( -45.49638112859755523, -291.0764482653454479, -344.3531133248914102 ) ) ;
#91313=CARTESIAN_POINT ( 'NONE',  ( 36.97648645787506183, -294.9389158397447090, -253.4727261746196234 ) ) ;
#91314=CARTESIAN_POINT ( 'NONE',  ( 201.3748867796775528, 292.7342570268831992, -53.99999999997705658 ) ) ;
#91316=CARTESIAN_POINT ( 'NONE',  ( -10.67920029253470204, -289.3465400325216592, -338.4815843186699453 ) ) ;
#91318=CARTESIAN_POINT ( 'NONE',  ( -111.4915245893550804, -296.9480044736803848, -290.7355215118308251 ) ) ;
#91319=CARTESIAN_POINT ( 'NONE',  ( -70.33802008173235265, -289.7614756711588484, -202.1588573561230362 ) ) ;
#91320=CARTESIAN_POINT ( 'NONE',  ( -35.47680861834266608, -298.4081822115830391, -193.3821595793300787 ) ) ;
#91323=CARTESIAN_POINT ( 'NONE',  ( -51.53717440752282641, -290.7506691636865526, -345.3357554339218041 ) ) ;
#91324=CARTESIAN_POINT ( 'NONE',  ( 13.79469577742117714, -283.1948066931273615, -206.1857440867352693 ) ) ;
#91325=CARTESIAN_POINT ( 'NONE',  ( -3.694709121519613504, -279.8330995285274412, -201.2004483965756094 ) ) ;
#91326=CARTESIAN_POINT ( 'NONE',  ( -70.82503165676855872, -287.6096530861794349, -203.4222750548792362 ) ) ;
#91327=CARTESIAN_POINT ( 'NONE',  ( 34.30806571156131923, -285.7886311819240746, -243.8108383795934913 ) ) ;
#91328=CARTESIAN_POINT ( 'NONE',  ( -70.27541464969006313, -271.6169354844466852, -203.1644002145726233 ) ) ;
#91329=CARTESIAN_POINT ( 'NONE',  ( -65.12857643057765245, -275.6064080204309334, -201.2879484714622436 ) ) ;
#91330=CARTESIAN_POINT ( 'NONE',  ( -105.3735108725226155, -288.2316181851806505, -300.7041839076871383 ) ) ;
#91331=CARTESIAN_POINT ( 'NONE',  ( -95.19049134432600567, -279.7423914618739786, -319.3078431985452994 ) ) ;
#91333=CARTESIAN_POINT ( 'NONE',  ( -27.55837506603365483, -280.1797575460331586, -197.9684690198365615 ) ) ;
#91334=CARTESIAN_POINT ( 'NONE',  ( 25.22782187993439962, -280.3799719185362278, -232.4615809328921614 ) ) ;
#91335=CARTESIAN_POINT ( 'NONE',  ( 36.20096867460583212, -276.9062808670003051, -292.1553155748598556 ) ) ;
#91336=CARTESIAN_POINT ( 'NONE',  ( 39.22244748885121624, -280.3777167532342673, -272.7983330314016257 ) ) ;
#91337=CARTESIAN_POINT ( 'NONE',  ( 159.3109176245238245, 219.1064649780328750, -202.8775829912029280 ) ) ;
#91338=CARTESIAN_POINT ( 'NONE',  ( 38.25828488781869652, -276.3253445144696343, -256.9645685401634978 ) ) ;
#91339=CARTESIAN_POINT ( 'NONE',  ( -36.91930833898076969, -299.4826080567211761, -193.9502423678791558 ) ) ;
#91340=CARTESIAN_POINT ( 'NONE',  ( 21.31550574532285580, -284.6948066931273615, -317.0979686699210447 ) ) ;
#91345=CARTESIAN_POINT ( 'NONE',  ( 8.182605621984954780, -289.4920466269820167, -327.8220930752488016 ) ) ;
#91346=CARTESIAN_POINT ( 'NONE',  ( 37.55421881697458986, -289.1487409091860172, -257.4560094781718931 ) ) ;
#91347=CARTESIAN_POINT ( 'NONE',  ( -109.5210734596103492, -289.7471891699900652, -282.0170710087725183 ) ) ;
#91348=CARTESIAN_POINT ( 'NONE',  ( -78.48425815463491517, -285.0216988905369817, -205.3471439294624759 ) ) ;
#91349=CARTESIAN_POINT ( 'NONE',  ( -21.01072962688938617, -108.8955080185006210, -362.6946229046635040 ) ) ;
#91350=CARTESIAN_POINT ( 'NONE',  ( 35.12362110089673450, -279.7688346066968279, -256.3224183162952272 ) ) ;
#91351=CARTESIAN_POINT ( 'NONE',  ( 34.21367010567445988, -289.1557266186640049, -250.5951251473379386 ) ) ;
#91352=CARTESIAN_POINT ( 'NONE',  ( -26.66124085334093152, -281.3938430229496817, -343.3281659134847246 ) ) ;
#91353=CARTESIAN_POINT ( 'NONE',  ( -110.3922834572073839, -279.7559256732691324, -278.8633887699262459 ) ) ;
#91354=AXIS2_PLACEMENT_3D ( 'NONE', #26901, #61504, #25491 ) ;
#91355=CARTESIAN_POINT ( 'NONE',  ( 0.9089829729819068893, -277.0195155218212335, -332.6690506112148000 ) ) ;
#91356=CARTESIAN_POINT ( 'NONE',  ( -113.9712288262322346, -289.3723632383288873, -268.3497450973521268 ) ) ;
#91357=CARTESIAN_POINT ( 'NONE',  ( -71.00473057962327061, -286.4220070058735814, -201.2889875521412932 ) ) ;
#91358=CARTESIAN_POINT ( 'NONE',  ( -113.7592462846896098, -285.1563676991896727, -261.4232467280049832 ) ) ;
#91359=CARTESIAN_POINT ( 'NONE',  ( 35.42920495873281794, -281.8031003738838649, -276.7490280684600634 ) ) ;
#91362=CARTESIAN_POINT ( 'NONE',  ( -111.4370641330658884, -292.6143455651869658, -254.4826574411059994 ) ) ;
#91364=CARTESIAN_POINT ( 'NONE',  ( -92.44519403408897062, -289.9689683647503671, -217.2112604745847761 ) ) ;
#91366=CARTESIAN_POINT ( 'NONE',  ( 34.12023193887684869, -274.8222826603795852, -286.4368627690673748 ) ) ;
#91367=CARTESIAN_POINT ( 'NONE',  ( -66.89294582374272125, -294.7779473027160293, -341.3685172502521255 ) ) ;
#91368=CARTESIAN_POINT ( 'NONE',  ( -32.08872379525112706, -290.5994559305301550, -196.8425005282266795 ) ) ;
#91369=CARTESIAN_POINT ( 'NONE',  ( 16.88654316452136683, -292.5061405806956714, -320.7324554999404995 ) ) ;
#91370=CARTESIAN_POINT ( 'NONE',  ( -90.87189489401639264, -291.0378026248541232, -320.6513421059987650 ) ) ;
#91372=AXIS2_PLACEMENT_3D ( 'NONE', #42228, #33269, #27109 ) ;
#91373=CARTESIAN_POINT ( 'NONE',  ( -70.98585459882744431, -291.4962940501667958, -337.3914955929608368 ) ) ;
#91374=CARTESIAN_POINT ( 'NONE',  ( 37.61481403398626355, -291.4800287185485104, -264.7442319228222800 ) ) ;
#91375=CARTESIAN_POINT ( 'NONE',  ( 34.76391171601918728, -295.2862059498849590, -249.6808263262046523 ) ) ;
#91376=CARTESIAN_POINT ( 'NONE',  ( -79.45434985963177610, -286.4093413322513015, -210.3828023599744483 ) ) ;
#91377=CARTESIAN_POINT ( 'NONE',  ( -50.12994296856311394, -297.2150176951487310, -344.4846158138618648 ) ) ;
#91379=CARTESIAN_POINT ( 'NONE',  ( 27.08296080288267405, -277.0094941831310962, -231.1734411330798480 ) ) ;
#91380=CARTESIAN_POINT ( 'NONE',  ( 23.19477141265485187, -274.9773544239545231, -317.3221813760087571 ) ) ;
#91382=CARTESIAN_POINT ( 'NONE',  ( -37.59684428451090810, -297.2462054656445503, -193.5230172586575463 ) ) ;
#91383=CARTESIAN_POINT ( 'NONE',  ( 12.41255121800860195, -274.5880988281972463, -325.2256112020459682 ) ) ;
#91384=CARTESIAN_POINT ( 'NONE',  ( -84.32809708462389153, -277.4801400354160705, -212.5571462392275350 ) ) ;
#91385=CARTESIAN_POINT ( 'NONE',  ( -38.10178674089300443, -275.2474962233858378, -196.9679795125657620 ) ) ;
#91386=CARTESIAN_POINT ( 'NONE',  ( 35.17655009341229544, -273.8195672833140861, -246.1170485126670258 ) ) ;
#91388=CARTESIAN_POINT ( 'NONE',  ( -50.55936929982452455, -296.6495469438519876, -342.7535771014049146 ) ) ;
#91390=CARTESIAN_POINT ( 'NONE',  ( -91.97226346387476781, -298.0492980665790697, -221.6979565887256456 ) ) ;
#91391=CARTESIAN_POINT ( 'NONE',  ( 144.2857639756989272, -299.5541904835127980, -189.7068768330456123 ) ) ;
#91392=CARTESIAN_POINT ( 'NONE',  ( 15.51390208675261206, -286.3298282326177855, -324.1429823475340299 ) ) ;
#91393=CARTESIAN_POINT ( 'NONE',  ( -109.8855308749134565, -272.4929590503043073, -262.2129510063363114 ) ) ;
#91394=CARTESIAN_POINT ( 'NONE',  ( -4.773947465373244547, -286.4693557288148895, -200.5876166622115306 ) ) ;
#91395=CARTESIAN_POINT ( 'NONE',  ( -34.67180554375087809, -288.6861812110296910, -347.2936595661045658 ) ) ;
#91396=CARTESIAN_POINT ( 'NONE',  ( -102.4418378916558368, -299.0378136671908464, -232.3059051094763845 ) ) ;
#91397=CARTESIAN_POINT ( 'NONE',  ( -53.57119342235846915, -293.2605465335681174, -343.4666668331450410 ) ) ;
#91398=CARTESIAN_POINT ( 'NONE',  ( 29.15197281433721344, -280.2475261933602724, -231.8546214042688121 ) ) ;
#91400=CARTESIAN_POINT ( 'NONE',  ( -85.83314923546242881, -277.3809199723460779, -213.0785918205089331 ) ) ;
#91402=CARTESIAN_POINT ( 'NONE',  ( -8.074190450822188225, -287.4550872398936576, -337.7247563930061460 ) ) ;
#91404=CARTESIAN_POINT ( 'NONE',  ( -45.60749175891414353, -287.1567656726519431, -344.9042419878641113 ) ) ;
#91405=CARTESIAN_POINT ( 'NONE',  ( -88.69691714495186829, -298.9172910876927745, -217.2889761594862534 ) ) ;
#91406=CARTESIAN_POINT ( 'NONE',  ( -3.140170789521716355, -284.0345894978480601, -338.7047296111546189 ) ) ;
#91407=CARTESIAN_POINT ( 'NONE',  ( -36.53656519700641070, -296.0822964683450209, -195.0061795729632479 ) ) ;
#91408=CARTESIAN_POINT ( 'NONE',  ( 35.51986069168074778, -281.4928733653972586, -265.8674607962465188 ) ) ;
#91409=CARTESIAN_POINT ( 'NONE',  ( -29.94857384365038655, -275.5728354481232714, -197.1442032660336565 ) ) ;
#91410=CARTESIAN_POINT ( 'NONE',  ( 35.74521643761639211, -285.8765823952537062, -289.5344543542438487 ) ) ;
#91411=CARTESIAN_POINT ( 'NONE',  ( -3.320735039392577637, -282.5014870460266252, -203.5068572701394203 ) ) ;
#91413=CARTESIAN_POINT ( 'NONE',  ( -92.24055986044469080, -272.1637059934034255, -221.7777743942119741 ) ) ;
#91416=CARTESIAN_POINT ( 'NONE',  ( -3.230692910975983878, -294.4474816213648865, -339.4078823316145872 ) ) ;
#91417=CARTESIAN_POINT ( 'NONE',  ( -102.4377971812799473, -287.0220629819997953, -233.7264399450374128 ) ) ;
#91419=CARTESIAN_POINT ( 'NONE',  ( -115.3430155898818299, -281.8380690714489560, -288.1317622949166548 ) ) ;
#91420=CARTESIAN_POINT ( 'NONE',  ( -99.52511600978857587, -277.1489645395939192, -315.5208588358211728 ) ) ;
#91421=CARTESIAN_POINT ( 'NONE',  ( -65.17400966114645655, -287.8095927481670628, -341.3520853129774082 ) ) ;
#91422=CARTESIAN_POINT ( 'NONE',  ( -76.47909747796536806, -285.1057547709830260, -332.8632061046549779 ) ) ;
#91423=CARTESIAN_POINT ( 'NONE',  ( -36.43153153290948865, -278.8007696303426428, -344.3814981817356511 ) ) ;
#91424=CARTESIAN_POINT ( 'NONE',  ( -110.1187585382362073, -285.6819420671899366, -293.6874052234516626 ) ) ;
#91425=CARTESIAN_POINT ( 'NONE',  ( -29.41695064357652356, -281.7445980916448889, -343.3798948244461258 ) ) ;
#91426=CARTESIAN_POINT ( 'NONE',  ( -71.88488443299729624, -281.5957443661278035, -203.7751089242213709 ) ) ;
#91427=CARTESIAN_POINT ( 'NONE',  ( -58.12365645485358812, -273.9576432399149439, -196.1631927018343049 ) ) ;
#91428=CARTESIAN_POINT ( 'NONE',  ( -111.4410944336392646, -278.1230939708128176, -291.2962503696851968 ) ) ;
#91429=CARTESIAN_POINT ( 'NONE',  ( -110.2910888526954238, -298.2797381086804194, -285.2468074337051007 ) ) ;
#91434=CARTESIAN_POINT ( 'NONE',  ( -109.6273850336243640, -294.9835581504654556, -247.4918916308654104 ) ) ;
#91435=CARTESIAN_POINT ( 'NONE',  ( 33.57042190436544615, -274.8278629516498199, -252.7696600922499499 ) ) ;
#91436=CARTESIAN_POINT ( 'NONE',  ( -109.7316728875863419, -274.0747173661319493, -245.3071649613955287 ) ) ;
#91437=CARTESIAN_POINT ( 'NONE',  ( 34.98149332624754493, -289.1076732822409099, -254.6343985227521500 ) ) ;
#91439=CARTESIAN_POINT ( 'NONE',  ( -33.45065499230291550, -296.5241534160896890, -346.5815171601796010 ) ) ;
#91440=CARTESIAN_POINT ( 'NONE',  ( 37.66993831308591467, -294.5611509607925314, -254.7642519674529353 ) ) ;
#91441=CARTESIAN_POINT ( 'NONE',  ( -91.91266301801832128, -291.8327591059735937, -321.6426059308977869 ) ) ;
#91442=CARTESIAN_POINT ( 'NONE',  ( -101.0145819251898018, -277.0820326412294321, -230.9457474183267323 ) ) ;
#91443=CARTESIAN_POINT ( 'NONE',  ( -109.0112319980739102, -280.7336544809712677, -250.1943641411609178 ) ) ;
#91444=CARTESIAN_POINT ( 'NONE',  ( -83.26705830995341273, -293.7662832120388998, -329.0116276548634460 ) ) ;
#91445=CARTESIAN_POINT ( 'NONE',  ( 8.480889543366975758, -284.2925163690293289, -330.6984675567716749 ) ) ;
#91447=CARTESIAN_POINT ( 'NONE',  ( -37.26680993935310227, -284.9734014890042886, -197.0395521222929176 ) ) ;
#91448=CARTESIAN_POINT ( 'NONE',  ( 162.9306247839069215, 218.7636628492012107, -204.5803896349958109 ) ) ;
#91449=ORIENTED_EDGE ( 'NONE', *, *, #22764, .T. ) ;
#91450=CARTESIAN_POINT ( 'NONE',  ( -68.78019434174719038, -285.2938222749552324, -204.4405076615336441 ) ) ;
#91452=CARTESIAN_POINT ( 'NONE',  ( 39.40104397242586742, -282.6262614602422332, -269.9182741761944726 ) ) ;
#91453=CARTESIAN_POINT ( 'NONE',  ( -107.9616278149003676, -273.1329137884198417, -251.5953418252914844 ) ) ;
#91454=CARTESIAN_POINT ( 'NONE',  ( -60.37582708712996293, -284.5550092692473640, -197.2480630011450558 ) ) ;
#91455=CARTESIAN_POINT ( 'NONE',  ( -2.507655499072967142, -281.4427498508011354, -201.9402264107646374 ) ) ;
#91456=CARTESIAN_POINT ( 'NONE',  ( -22.71818901303054616, -281.7560159376803313, -195.4150260402975334 ) ) ;
#91457=CARTESIAN_POINT ( 'NONE',  ( 23.66136972373545433, -281.5779690507591226, -223.5214694981244747 ) ) ;
#91458=CARTESIAN_POINT ( 'NONE',  ( -67.74223827176246004, -280.9809262143061233, -333.4151289067050357 ) ) ;
#91459=CARTESIAN_POINT ( 'NONE',  ( -89.20268650580214853, -231.0846910060161576, -347.9280380252721443 ) ) ;
#91460=ORIENTED_EDGE ( 'NONE', *, *, #89262, .F. ) ;
#91461=CARTESIAN_POINT ( 'NONE',  ( -91.54158464531045070, -275.2782973075043174, -218.7439046091689363 ) ) ;
#91462=CARTESIAN_POINT ( 'NONE',  ( -114.2130971324556441, -273.2892385179353028, -270.3705028573608615 ) ) ;
#91463=CARTESIAN_POINT ( 'NONE',  ( -107.0412691870660922, -276.9229084974386410, -243.4991220509693335 ) ) ;
#91464=CARTESIAN_POINT ( 'NONE',  ( -2.540179950329658709, -294.2661110412163907, -202.7978267517777908 ) ) ;
#91465=CARTESIAN_POINT ( 'NONE',  ( -66.10086824468920952, -294.7873696022830927, -337.5682821665109827 ) ) ;
#91466=CARTESIAN_POINT ( 'NONE',  ( -5.906338203719967872, -291.9620620304044110, -200.1233049616625124 ) ) ;
#91467=CARTESIAN_POINT ( 'NONE',  ( -88.01845085739296337, -229.9137135291527159, -344.5856900492037767 ) ) ;
#91468=CARTESIAN_POINT ( 'NONE',  ( -113.1876926100662075, -295.2437508701562479, -261.0879461010388241 ) ) ;
#91469=CARTESIAN_POINT ( 'NONE',  ( 28.93739615278737531, -286.3869320849117344, -302.8191186786874596 ) ) ;
#91470=CARTESIAN_POINT ( 'NONE',  ( 18.92387230723247171, -296.0908895032135320, -318.8062327677308190 ) ) ;
#91471=CARTESIAN_POINT ( 'NONE',  ( 36.17413427506936330, -286.2101645750043986, -268.3153303142756840 ) ) ;
#91472=CARTESIAN_POINT ( 'NONE',  ( -85.17011665110520369, -285.0442949659156966, -326.1615306116070201 ) ) ;
#91474=CARTESIAN_POINT ( 'NONE',  ( -47.72347311982773022, -292.8646121133641032, -194.2480429103480333 ) ) ;
#91475=CARTESIAN_POINT ( 'NONE',  ( -51.02327871930491199, -283.7239513089365914, -342.1818311753037278 ) ) ;
#91476=CARTESIAN_POINT ( 'NONE',  ( -113.9694323779194605, -295.3208984764758611, -272.4436056596489948 ) ) ;
#91477=CARTESIAN_POINT ( 'NONE',  ( -111.8405351030341848, -291.5915210528933130, -251.4910140995811787 ) ) ;
#91478=CARTESIAN_POINT ( 'NONE',  ( -25.03746414870094128, -292.6973995371104706, -194.4128943032258690 ) ) ;
#91479=CARTESIAN_POINT ( 'NONE',  ( 28.80905960562859747, -287.3019639123954789, -239.4891729331150714 ) ) ;
#91482=CARTESIAN_POINT ( 'NONE',  ( -81.13806443618545927, -297.5001987460254895, -332.2489965217478129 ) ) ;
#91483=CARTESIAN_POINT ( 'NONE',  ( -14.97251956371161263, -297.0115246069310615, -193.8591426424625865 ) ) ;
#91484=CARTESIAN_POINT ( 'NONE',  ( -71.03929899225272493, -278.6548075280031185, -205.3248338465427025 ) ) ;
#91485=CARTESIAN_POINT ( 'NONE',  ( 22.71425433338012212, -274.4148920279678237, -222.2485482977347715 ) ) ;
#91486=CARTESIAN_POINT ( 'NONE',  ( 1.538203921088562742, -278.3873637134157661, -333.6609051914350630 ) ) ;
#91487=CARTESIAN_POINT ( 'NONE',  ( 19.96727743928017063, -273.0341798151374064, -223.1748215228151935 ) ) ;
#91488=CARTESIAN_POINT ( 'NONE',  ( -10.32966836467748628, -295.8966728383643954, -338.6068551764698782 ) ) ;
#91489=CARTESIAN_POINT ( 'NONE',  ( -95.54283132745888452, -298.2564638759285458, -225.7665143323638972 ) ) ;
#91490=CARTESIAN_POINT ( 'NONE',  ( -47.50449942084240007, -296.7794073300615878, -345.8803733062347874 ) ) ;
#91491=CARTESIAN_POINT ( 'NONE',  ( -92.91484279393951340, -271.2798075829547884, -219.4497106490539693 ) ) ;
#91492=CARTESIAN_POINT ( 'NONE',  ( -33.51137945871451507, -292.7530184164127149, -197.3470924747991546 ) ) ;
#91493=CARTESIAN_POINT ( 'NONE',  ( -95.42676766480094841, -288.4951942623794707, -315.5644434295701899 ) ) ;
#91494=DIRECTION ( 'NONE',  ( 0.000000000000000000, 0.000000000000000000, 1.000000000000000000 ) ) ;
#91495=CARTESIAN_POINT ( 'NONE',  ( 36.52500573981465948, -275.7722603408423652, -248.6520603133711518 ) ) ;
#91496=CARTESIAN_POINT ( 'NONE',  ( -84.09162628998343791, -297.7223299358935833, -214.2011407828729261 ) ) ;
#91497=CARTESIAN_POINT ( 'NONE',  ( -61.54375299023272561, -281.7193171916490542, -198.9431522441431923 ) ) ;
#91498=CARTESIAN_POINT ( 'NONE',  ( 37.06481366238827491, -280.4617349392677284, -288.2205692750201251 ) ) ;
#91499=CARTESIAN_POINT ( 'NONE',  ( -70.26491466348439019, -276.8232310769152491, -339.8692397099854361 ) ) ;
#91500=CARTESIAN_POINT ( 'NONE',  ( -7.196263891439274474, -281.8434792663929898, -337.0371020368896779 ) ) ;
#91501=CARTESIAN_POINT ( 'NONE',  ( 8.080217619880164293, -280.4325612955711335, -330.2516665827125166 ) ) ;
#91503=CARTESIAN_POINT ( 'NONE',  ( 11.95459705568524456, -273.3277364390233402, -215.6550468585326712 ) ) ;
#91504=CARTESIAN_POINT ( 'NONE',  ( -6.857282316264694089, -278.6522482819830770, -338.9001472053624866 ) ) ;
#91506=DIRECTION ( 'NONE',  ( 1.000000000000000000, 0.000000000000000000, 0.000000000000000000 ) ) ;
#91507=CARTESIAN_POINT ( 'NONE',  ( -45.99197099733657979, -296.1837418153170916, -194.8684241207276955 ) ) ;
#91508=CARTESIAN_POINT ( 'NONE',  ( -109.4738409625824005, -290.8946200070876671, -243.2656314837360298 ) ) ;
#91509=CARTESIAN_POINT ( 'NONE',  ( 7.176259856942059479, -278.4478500041583402, -330.9910744772145108 ) ) ;
#91510=CARTESIAN_POINT ( 'NONE',  ( 21.43844668523864172, -272.9118451248900215, -223.7584271836043683 ) ) ;
#91512=CARTESIAN_POINT ( 'NONE',  ( -99.81985490410760065, -287.0443997037538111, -227.7740099923798027 ) ) ;
#91515=CARTESIAN_POINT ( 'NONE',  ( 17.49309829754145440, -286.2684429627485088, -321.5476067367169435 ) ) ;
#91517=CARTESIAN_POINT ( 'NONE',  ( -39.71718064777807200, -293.8775345210710270, -343.7322390492487330 ) ) ;
#91518=CARTESIAN_POINT ( 'NONE',  ( 23.00937639164871129, -285.0966077774099290, -227.0469595182767080 ) ) ;
#91520=CARTESIAN_POINT ( 'NONE',  ( -66.86320858918466570, -293.4388402704298642, -339.3066123174010613 ) ) ;
#91521=CARTESIAN_POINT ( 'NONE',  ( 15.83005975248296160, -285.2688731667498701, -215.6302153513252335 ) ) ;
#91522=CARTESIAN_POINT ( 'NONE',  ( -110.4168739231098044, -280.2915565306478811, -259.6879277718881553 ) ) ;
#91523=CARTESIAN_POINT ( 'NONE',  ( 29.77621589810125968, -288.2753172226339871, -233.3296375582851852 ) ) ;
#91524=CARTESIAN_POINT ( 'NONE',  ( 36.87094569955860379, -279.9996485591304349, -286.7446456762218077 ) ) ;
#91525=CARTESIAN_POINT ( 'NONE',  ( -66.32902935581385861, -289.4424156244938331, -337.4131546158085371 ) ) ;
#91526=CARTESIAN_POINT ( 'NONE',  ( -65.05470993436355798, -281.1080922550962669, -202.1895402891388756 ) ) ;
#91527=CARTESIAN_POINT ( 'NONE',  ( 11.40582208700768518, -281.5517825427929779, -215.8058175580083287 ) ) ;
#91528=CARTESIAN_POINT ( 'NONE',  ( -33.82975818805260815, -288.0760300475851636, -195.0877955600566622 ) ) ;
#91530=CARTESIAN_POINT ( 'NONE',  ( -15.77735919573738954, -274.3235032201508261, -196.3870452591940250 ) ) ;
#91531=CARTESIAN_POINT ( 'NONE',  ( -108.1391329845408222, -292.8392824673886139, -246.7058795961908118 ) ) ;
#91533=CARTESIAN_POINT ( 'NONE',  ( -112.3452863284742875, -275.1604526064900824, -261.9424758988611188 ) ) ;
#91535=CARTESIAN_POINT ( 'NONE',  ( -4.601070507658654662, -272.4822888427931957, -202.6854445685419819 ) ) ;
#91537=CARTESIAN_POINT ( 'NONE',  ( -76.68680171292136549, -293.9689646864444512, -335.6789566600926946 ) ) ;
#91538=CARTESIAN_POINT ( 'NONE',  ( -104.8166454803574794, -296.4352407168179866, -242.3411217084400562 ) ) ;
#91540=CARTESIAN_POINT ( 'NONE',  ( -3.026432016498052491, -290.1106147667691744, -335.6339768666276200 ) ) ;
#91541=CARTESIAN_POINT ( 'NONE',  ( 14.65228333007634554, -284.0684307898442285, -323.1077696386612388 ) ) ;
#91542=CARTESIAN_POINT ( 'NONE',  ( -54.35264091286074262, -290.6916595935194891, -344.9085905796628140 ) ) ;
#91543=CARTESIAN_POINT ( 'NONE',  ( -111.1614163470662504, -292.1212322598742617, -250.2129138352427447 ) ) ;
#91544=CARTESIAN_POINT ( 'NONE',  ( -98.21256529863494222, -287.1488889457705227, -226.5243796244758130 ) ) ;
#91545=CARTESIAN_POINT ( 'NONE',  ( -59.30417266740785465, -279.9421459336763860, -196.5596965568990981 ) ) ;
#91546=CARTESIAN_POINT ( 'NONE',  ( -85.49675451179396646, -293.7919961329496346, -328.5883017756792128 ) ) ;
#91547=CARTESIAN_POINT ( 'NONE',  ( -74.27785059713075100, -283.3621963305916438, -337.9833280790210779 ) ) ;
#91548=CARTESIAN_POINT ( 'NONE',  ( 28.95392921547570708, -276.9667457095656005, -236.9581988374690411 ) ) ;
#91549=CARTESIAN_POINT ( 'NONE',  ( 31.03373250439201669, -301.4082689599840705, -195.3320873922940848 ) ) ;
#91550=CARTESIAN_POINT ( 'NONE',  ( 14.17943005956878189, -274.5805609200348840, -326.2856185780856890 ) ) ;
#91552=CARTESIAN_POINT ( 'NONE',  ( 25.60887001799556728, -281.5699379870615076, -307.5449553459628760 ) ) ;
#91553=CARTESIAN_POINT ( 'NONE',  ( -71.38054830402484185, -278.6967495891598787, -338.9859351782491785 ) ) ;
#91554=CARTESIAN_POINT ( 'NONE',  ( -36.55576499275309033, -285.1205429722402869, -193.5874352143536612 ) ) ;
#91555=CARTESIAN_POINT ( 'NONE',  ( -73.13641183575981586, -293.3313159366523450, -205.5214786443138451 ) ) ;
#91556=CARTESIAN_POINT ( 'NONE',  ( -102.0505484084054046, -274.6842044202846296, -230.1217669854655128 ) ) ;
#91557=CARTESIAN_POINT ( 'NONE',  ( -78.58985866657772590, -274.8242253368149477, -205.9259747048038491 ) ) ;
#91559=CARTESIAN_POINT ( 'NONE',  ( -6.278554105478609593, -276.4656431564644663, -336.4360772835125317 ) ) ;
#91560=CARTESIAN_POINT ( 'NONE',  ( -111.8787855641530484, -298.6451428517201521, -263.1476459874509715 ) ) ;
#91561=CARTESIAN_POINT ( 'NONE',  ( -69.54127732539646445, -283.6272128542339033, -202.7954072085723283 ) ) ;
#91562=CARTESIAN_POINT ( 'NONE',  ( 26.47775162097885016, -292.6504917385881299, -227.2229252906625163 ) ) ;
#91563=CARTESIAN_POINT ( 'NONE',  ( 12.83511596333008775, -274.3683832450362274, -325.6954536688811572 ) ) ;
#91564=CARTESIAN_POINT ( 'NONE',  ( -37.47947447601243454, -290.6539350619147513, -346.5739325317918542 ) ) ;
#91566=CARTESIAN_POINT ( 'NONE',  ( 13.12587306266063081, -291.6981549386446773, -217.1892256963067211 ) ) ;
#91568=CARTESIAN_POINT ( 'NONE',  ( -41.99977039435461990, -290.5692526024471363, -194.0924568252665949 ) ) ;
#91569=CARTESIAN_POINT ( 'NONE',  ( -106.0539009480764321, -289.8898351486674869, -295.0738868522901157 ) ) ;
#91571=CARTESIAN_POINT ( 'NONE',  ( 30.09744879894085301, -289.1073502841383629, -306.9887024118148702 ) ) ;
#91572=CARTESIAN_POINT ( 'NONE',  ( -93.95961154558501960, -279.5379800872693181, -224.2471331884474353 ) ) ;
#91574=CARTESIAN_POINT ( 'NONE',  ( -79.31930809994936737, -294.5249612173482205, -334.5434593091197826 ) ) ;
#91575=CARTESIAN_POINT ( 'NONE',  ( -10.03792312476201332, -287.0507189585259198, -198.4168679114301597 ) ) ;
#91576=CARTESIAN_POINT ( 'NONE',  ( -113.4671669276836781, -285.0328249901880895, -258.5789369413884060 ) ) ;
#91577=CARTESIAN_POINT ( 'NONE',  ( -32.13996031343946669, -283.3180107188272245, -343.1967506749186327 ) ) ;
#91578=CARTESIAN_POINT ( 'NONE',  ( -110.2157014284088206, -266.9174177228133544, -307.0198616398569129 ) ) ;
#91579=CARTESIAN_POINT ( 'NONE',  ( -108.4223761982444358, -261.1587273596273349, -317.0417516531400679 ) ) ;
#91580=CARTESIAN_POINT ( 'NONE',  ( -63.66200778950266681, -182.2673717872931718, -358.7378838168659740 ) ) ;
#91581=CARTESIAN_POINT ( 'NONE',  ( 11.66224941634359702, -273.9500759587870107, -215.9678109672791493 ) ) ;
#91582=CARTESIAN_POINT ( 'NONE',  ( 9.852595745083579715, -275.3043725013017706, -326.4585734480855876 ) ) ;
#91583=CARTESIAN_POINT ( 'NONE',  ( -100.6964262628418822, -296.6368665958761426, -226.6835801233826544 ) ) ;
#91584=CARTESIAN_POINT ( 'NONE',  ( 190.0960685029364186, 268.0118023413412516, -137.8165032444274232 ) ) ;
#91585=CARTESIAN_POINT ( 'NONE',  ( 36.01581549171817187, -274.5118220894777892, -292.1322483152757172 ) ) ;
#91586=CARTESIAN_POINT ( 'NONE',  ( -108.9258722442364586, -274.5595422837134834, -251.3579791469701092 ) ) ;
#91588=CARTESIAN_POINT ( 'NONE',  ( -85.07949011988362997, -298.3525370706499871, -210.2451997996368789 ) ) ;
#91590=CARTESIAN_POINT ( 'NONE',  ( -31.86048534033557189, -289.4736123481187064, -343.2674270434939103 ) ) ;
#91591=PRODUCT_DEFINITION ( 'UNKNOWN', '', #62834, #28627 ) ;
#91592=CARTESIAN_POINT ( 'NONE',  ( -39.09388820444630142, -295.8764454847183742, -347.1796616945701999 ) ) ;
#91593=CARTESIAN_POINT ( 'NONE',  ( -99.04684290866012475, -297.6564628810481281, -224.3826016525354987 ) ) ;
#91594=CARTESIAN_POINT ( 'NONE',  ( -17.43463496833863857, -292.4828236523838996, -200.0752807098855612 ) ) ;
#91596=CARTESIAN_POINT ( 'NONE',  ( 38.26673009654518154, -277.4821339957850341, -271.1320804500407462 ) ) ;
#91598=CARTESIAN_POINT ( 'NONE',  ( 19.11926616122301681, -280.3473024399932569, -218.0955825990215544 ) ) ;
#91599=CARTESIAN_POINT ( 'NONE',  ( -21.59077009152522919, -277.7866273271833961, -341.9347218537813546 ) ) ;
#91600=CARTESIAN_POINT ( 'NONE',  ( -1.919964192950602166, -278.3496514733835738, -337.5866684754669791 ) ) ;
#91601=CARTESIAN_POINT ( 'NONE',  ( -112.1369473547592008, -276.4497868026714968, -279.9447579437610329 ) ) ;
#91602=CARTESIAN_POINT ( 'NONE',  ( -79.79397176477503706, -298.1122816857189264, -210.8489570339458226 ) ) ;
#91603=CARTESIAN_POINT ( 'NONE',  ( -104.2467940553128471, -295.5383155970454254, -239.5940671088083889 ) ) ;
#91605=CARTESIAN_POINT ( 'NONE',  ( -68.65322629069373761, -280.1439077479072921, -200.0679039868539917 ) ) ;
#91606=CARTESIAN_POINT ( 'NONE',  ( -99.17396301451606178, -278.1818461641130966, -309.2598048186122242 ) ) ;
#91608=CARTESIAN_POINT ( 'NONE',  ( 0.4609520040583713896, -287.2445834700441765, -336.9360728893208830 ) ) ;
#91609=CARTESIAN_POINT ( 'NONE',  ( -36.24417668106679002, -300.0660164118279454, -195.1940694812736581 ) ) ;
#91611=CARTESIAN_POINT ( 'NONE',  ( -29.16520366839402101, -288.1430477874945382, -343.0642584406153901 ) ) ;
#91612=CARTESIAN_POINT ( 'NONE',  ( -67.70174011012508686, -277.8880789417145252, -202.8473845359850145 ) ) ;
#91613=CARTESIAN_POINT ( 'NONE',  ( -96.87176147297223849, -277.7275030896753378, -227.0997412772513542 ) ) ;
#91614=CARTESIAN_POINT ( 'NONE',  ( -48.56954327302700136, -281.2760509465280734, -343.9494984108547442 ) ) ;
#91615=CARTESIAN_POINT ( 'NONE',  ( 7.727946979128574867, -288.6671836073599593, -210.3491585421080856 ) ) ;
#91616=CARTESIAN_POINT ( 'NONE',  ( -106.8255794051055148, -280.0716171944793018, -246.5592039537742721 ) ) ;
#91618=CARTESIAN_POINT ( 'NONE',  ( 11.94451510271255223, -294.7373705039797187, -213.8290948968864313 ) ) ;
#91619=CARTESIAN_POINT ( 'NONE',  ( -112.0731805711758824, -276.6167981050014077, -284.1869860743988170 ) ) ;
#91620=CARTESIAN_POINT ( 'NONE',  ( 32.61634922327148445, -276.4845052686296185, -291.6121676816976560 ) ) ;
#91621=CARTESIAN_POINT ( 'NONE',  ( 31.48381616399933236, -283.1575354268622959, -240.1439584408999508 ) ) ;
#91622=ADVANCED_FACE ( 'NONE', ( #73766, #66211 ), #58638, .F. ) ;
#91625=CARTESIAN_POINT ( 'NONE',  ( -84.25118808361536082, -291.6113564657768507, -329.6631017887759185 ) ) ;
#91626=CARTESIAN_POINT ( 'NONE',  ( -66.51375320186078000, -293.4338849471275239, -339.5097269361399412 ) ) ;
#91627=CARTESIAN_POINT ( 'NONE',  ( -110.9562215495007109, -283.4718440125857342, -292.4309300503533109 ) ) ;
#91629=CARTESIAN_POINT ( 'NONE',  ( -72.12645278304323426, -272.2671343253006739, -205.5644431610330400 ) ) ;
#91630=CARTESIAN_POINT ( 'NONE',  ( -30.67280933041948998, -290.2769392037974399, -196.4260696246104203 ) ) ;
#91632=CARTESIAN_POINT ( 'NONE',  ( -73.09159571276958900, -290.0670039747904525, -202.9323145836915501 ) ) ;
#91633=CARTESIAN_POINT ( 'NONE',  ( -42.75290109789580839, -287.5829069618486074, -196.7469999284384414 ) ) ;
#91634=CARTESIAN_POINT ( 'NONE',  ( 33.91190192797236591, -285.4538162053688097, -243.9622883441582246 ) ) ;
#91635=CARTESIAN_POINT ( 'NONE',  ( -57.57366874214088881, -287.2112103157493266, -199.5546844910101356 ) ) ;
#91637=CARTESIAN_POINT ( 'NONE',  ( -103.6361057395393885, -285.7733673289069429, -239.2950097593211751 ) ) ;
#91638=CARTESIAN_POINT ( 'NONE',  ( 26.64214457312336748, -294.9988019725332720, -230.4571164693560945 ) ) ;
#91639=CARTESIAN_POINT ( 'NONE',  ( 37.50127350561799489, -273.4996481698258890, -259.9763456916354585 ) ) ;
#91640=CARTESIAN_POINT ( 'NONE',  ( 18.89066463898398851, -276.6026274741958559, -322.9316938232645384 ) ) ;
#91641=CARTESIAN_POINT ( 'NONE',  ( 5.696469485077396477, -290.7101971354200600, -208.2561250100925747 ) ) ;
#91642=CARTESIAN_POINT ( 'NONE',  ( -112.7936298316086976, -278.3592080234463424, -285.7887752910229437 ) ) ;
#91643=CARTESIAN_POINT ( 'NONE',  ( -35.58723491855735688, -297.0099543659138703, -344.9980781415468982 ) ) ;
#91645=DIRECTION ( 'NONE',  ( 0.000000000000000000, 0.000000000000000000, -1.000000000000000000 ) ) ;
#91646=CARTESIAN_POINT ( 'NONE',  ( -102.6691503550455593, -283.6916143707038600, -236.6926204891089185 ) ) ;
#91647=CARTESIAN_POINT ( 'NONE',  ( 20.44641471730726678, -278.8922418264461953, -222.5538545683616860 ) ) ;
#91649=CARTESIAN_POINT ( 'NONE',  ( -4.110393303378095275, -272.9622495973496257, -201.6562146196084484 ) ) ;
#91650=CARTESIAN_POINT ( 'NONE',  ( -71.70943302926131935, -276.8675170919686366, -334.8946273709447610 ) ) ;
#91652=CARTESIAN_POINT ( 'NONE',  ( -42.41834566421157859, -296.6374639314518049, -343.8793838968330761 ) ) ;
#91653=CARTESIAN_POINT ( 'NONE',  ( 32.89537836024536688, -280.0781992771161413, -239.5675258839310686 ) ) ;
#91654=CARTESIAN_POINT ( 'NONE',  ( 16.33974101785182853, -295.2070978176341214, -320.1778955255865071 ) ) ;
#91655=CARTESIAN_POINT ( 'NONE',  ( -16.62421798375591209, -296.1052394823257146, -344.0643831288477372 ) ) ;
#91656=CARTESIAN_POINT ( 'NONE',  ( -95.28777342368346126, -297.0103140906840622, -225.9419603996430226 ) ) ;
#91657=CARTESIAN_POINT ( 'NONE',  ( -110.3808649490486005, -292.7717898374029346, -253.2673950070856677 ) ) ;
#91658=CARTESIAN_POINT ( 'NONE',  ( -91.90448717070616169, -285.4661207114720582, -216.0297064912361691 ) ) ;
#91659=CARTESIAN_POINT ( 'NONE',  ( -8.379090772105486806, -274.8166112892657225, -340.3856901209849752 ) ) ;
#91660=CARTESIAN_POINT ( 'NONE',  ( -34.66894647719743716, -288.8527554178075434, -347.3147169396272602 ) ) ;
#91661=CARTESIAN_POINT ( 'NONE',  ( -16.48578085765428369, -282.3028996450793784, -198.6891050937911984 ) ) ;
#91662=CARTESIAN_POINT ( 'NONE',  ( 20.53394647460082822, -285.9808768801356109, -225.4855346527272673 ) ) ;
#91663=CARTESIAN_POINT ( 'NONE',  ( -63.66242236807559607, -289.7090353403514769, -200.0766450495821687 ) ) ;
#91664=CARTESIAN_POINT ( 'NONE',  ( 202.1133578493929974, 280.9843981858382449, -111.1516734208197050 ) ) ;
#91665=CARTESIAN_POINT ( 'NONE',  ( -5.766379998217369796, -285.9864818107648148, -204.4611503838049771 ) ) ;
#91667=CARTESIAN_POINT ( 'NONE',  ( -16.19511271854763024, -283.7266386584992688, -344.2108313378158186 ) ) ;
#91668=CARTESIAN_POINT ( 'NONE',  ( -64.29492612794344097, -290.7677730558818894, -198.4278374441607582 ) ) ;
#91669=CARTESIAN_POINT ( 'NONE',  ( 38.00056594634853724, -283.0038771750467390, -258.6184678580630134 ) ) ;
#91670=CARTESIAN_POINT ( 'NONE',  ( -110.9613867094538904, -279.6047086496683960, -291.1803403766498946 ) ) ;
#91671=CARTESIAN_POINT ( 'NONE',  ( 35.35255650702463726, -281.2903900979920877, -263.1534556928802999 ) ) ;
#91672=CARTESIAN_POINT ( 'NONE',  ( -16.09790370714123497, -276.3268667571045398, -198.3785230062812843 ) ) ;
#91673=CARTESIAN_POINT ( 'NONE',  ( -70.80787226600439510, -295.4813837412916087, -339.7226923413282975 ) ) ;
#91674=CARTESIAN_POINT ( 'NONE',  ( -84.85707358039164205, -289.4131982856992522, -212.7925841703364824 ) ) ;
#91676=CARTESIAN_POINT ( 'NONE',  ( -65.67956025985559165, -296.5929058063541106, -202.7505288912029755 ) ) ;
#91677=ORIENTED_EDGE ( 'NONE', *, *, #61610, .F. ) ;
#91678=CARTESIAN_POINT ( 'NONE',  ( -96.93311372400863490, -287.0863581395156530, -225.7497110762313639 ) ) ;
#91680=CARTESIAN_POINT ( 'NONE',  ( -37.80700652970080711, -293.1261177018325839, -193.6716402084201718 ) ) ;
#91681=CARTESIAN_POINT ( 'NONE',  ( -69.04587751631092374, -284.1319044414154860, -336.2440352460590702 ) ) ;
#91682=CARTESIAN_POINT ( 'NONE',  ( 9.376661853561191862, -273.7355459901817767, -209.4495848706881134 ) ) ;
#91683=CARTESIAN_POINT ( 'NONE',  ( -104.5249557294449971, -291.6892164454312137, -232.9482464927356489 ) ) ;
#91684=CARTESIAN_POINT ( 'NONE',  ( -106.7843600063659864, -283.0858162600539458, -239.9311469303197271 ) ) ;
#91685=CARTESIAN_POINT ( 'NONE',  ( -30.70332401068005623, -292.4670464085056665, -193.6162868816578850 ) ) ;
#91686=CARTESIAN_POINT ( 'NONE',  ( 31.85927862664286181, -287.5758766648709752, -247.0520633868182756 ) ) ;
#91688=CARTESIAN_POINT ( 'NONE',  ( -97.78953360390984528, -246.5544654070388901, -331.3250685880491915 ) ) ;
#91689=CARTESIAN_POINT ( 'NONE',  ( 11.06782603903197781, -283.9164310913357667, -329.4144678386594478 ) ) ;
#91690=CARTESIAN_POINT ( 'NONE',  ( 31.98288692825983404, -284.6237833571634042, -237.0123917617631264 ) ) ;
#91692=CARTESIAN_POINT ( 'NONE',  ( 29.25923994371089876, -280.0594779340414107, -239.6037990337738108 ) ) ;
#91693=CARTESIAN_POINT ( 'NONE',  ( -42.80890441612591957, -276.7860923562897710, -347.1455823539620837 ) ) ;
#91694=CARTESIAN_POINT ( 'NONE',  ( -32.87849668878786247, -282.1086894124832725, -195.6609958751906220 ) ) ;
#91695=CARTESIAN_POINT ( 'NONE',  ( 66.77714209949721180, 46.10201122810671137, -317.1972835727068514 ) ) ;
#91696=CARTESIAN_POINT ( 'NONE',  ( 33.78266960039268696, -279.7684819353552825, -242.2893835750898006 ) ) ;
#91697=CARTESIAN_POINT ( 'NONE',  ( -104.9651022474555049, -282.9910903011765413, -238.6329437063494936 ) ) ;
#91698=CARTESIAN_POINT ( 'NONE',  ( -59.86933866991501674, -299.5244753058009337, -197.7358065938024936 ) ) ;
#91699=CARTESIAN_POINT ( 'NONE',  ( 21.03919886363193115, -293.4281445012146037, -226.4332330488559535 ) ) ;
#91700=ORIENTED_EDGE ( 'NONE', *, *, #61930, .F. ) ;
#91701=CARTESIAN_POINT ( 'NONE',  ( -110.8303546302146430, -289.2263167016748753, -271.1742207043170083 ) ) ;
#91702=CARTESIAN_POINT ( 'NONE',  ( 39.52192656842822771, -276.2495196040169958, -274.0308160220959621 ) ) ;
#91703=CARTESIAN_POINT ( 'NONE',  ( -35.81771388425057268, -298.2384338344615458, -197.3610733349210307 ) ) ;
#91705=CARTESIAN_POINT ( 'NONE',  ( -7.796899972571944559, -273.3505533472036291, -199.5332986406163229 ) ) ;
#91706=CARTESIAN_POINT ( 'NONE',  ( 144.2857639756989272, -299.5541904835127980, -201.0153591320744226 ) ) ;
#91709=CARTESIAN_POINT ( 'NONE',  ( 16.06043083789317194, -283.3524651980815179, -320.6582549383179526 ) ) ;
#91710=CARTESIAN_POINT ( 'NONE',  ( 23.45795931788408950, -283.9269596676531933, -315.9393521227596580 ) ) ;
#91711=CARTESIAN_POINT ( 'NONE',  ( -101.9845361584891776, -283.1420753304184927, -304.8887313686983020 ) ) ;
#91712=CARTESIAN_POINT ( 'NONE',  ( 23.72564104763106130, -273.3817406380417196, -228.8990854082144892 ) ) ;
#91713=CARTESIAN_POINT ( 'NONE',  ( 36.75126273659486742, -283.3529897628757794, -265.7678259215918501 ) ) ;
#91714=CARTESIAN_POINT ( 'NONE',  ( 34.83980279765318500, -274.2260877448811129, -285.2116529775123581 ) ) ;
#91716=CARTESIAN_POINT ( 'NONE',  ( 35.41461877289251703, -276.7551922408595715, -279.7523525690032784 ) ) ;
#91718=CARTESIAN_POINT ( 'NONE',  ( -112.6333464956169905, -279.1619107544272538, -285.7664656497231022 ) ) ;
#91722=CARTESIAN_POINT ( 'NONE',  ( -111.3138993237154040, -286.2043231567379848, -286.7446228228934046 ) ) ;
#91724=CARTESIAN_POINT ( 'NONE',  ( -6.706584450672058217, -293.8365004650218566, -336.7997469187502588 ) ) ;
#91725=CARTESIAN_POINT ( 'NONE',  ( -3.113565606788212481, -287.9605343500850836, -339.2360750304758881 ) ) ;
#91726=CARTESIAN_POINT ( 'NONE',  ( -44.09482455433020220, -284.2054497223587646, -196.6565094170741190 ) ) ;
#91727=CARTESIAN_POINT ( 'NONE',  ( -109.0032193232709687, -282.9072508542182049, -287.1494823584988580 ) ) ;
#91728=CARTESIAN_POINT ( 'NONE',  ( -64.20936656575456425, -287.6472766143098738, -339.3805644166588991 ) ) ;
#91729=CARTESIAN_POINT ( 'NONE',  ( -108.1401275136907998, -285.5023079593642592, -289.7660414748662561 ) ) ;
#91730=CARTESIAN_POINT ( 'NONE',  ( 13.50798406253006334, -274.3405802992307940, -325.5617193760199939 ) ) ;
#91731=CARTESIAN_POINT ( 'NONE',  ( 4.754873096778361230, -285.0098494613138200, -206.7819721037364502 ) ) ;
#91732=CARTESIAN_POINT ( 'NONE',  ( -110.6511567924562485, -298.7563420412542996, -254.4668045767008948 ) ) ;
#91733=CARTESIAN_POINT ( 'NONE',  ( -111.6705326620546970, -282.6997599140643160, -258.8270086063118356 ) ) ;
#91734=CARTESIAN_POINT ( 'NONE',  ( 29.18140896738806589, -282.0800761637487426, -239.6114658502153532 ) ) ;
#91735=CARTESIAN_POINT ( 'NONE',  ( -8.902587315481309105, -290.6812121743489001, -339.9541046579662975 ) ) ;
#91739=CARTESIAN_POINT ( 'NONE',  ( -96.26876338466560412, -297.8262628224761102, -317.6776274099951252 ) ) ;
#91740=CARTESIAN_POINT ( 'NONE',  ( -35.59126679820413131, -278.0739276898694925, -195.3688009783398059 ) ) ;
#91741=CARTESIAN_POINT ( 'NONE',  ( 22.98766303208299533, -292.1113056397780383, -222.7530447998403815 ) ) ;
#91742=CARTESIAN_POINT ( 'NONE',  ( -105.7106075919401889, -294.5838432640967994, -298.1483975485358542 ) ) ;
#91743=CARTESIAN_POINT ( 'NONE',  ( -77.07448203530071851, -278.1926744803297424, -208.4736902566769174 ) ) ;
#91744=CARTESIAN_POINT ( 'NONE',  ( -43.57887120726325492, -272.0527257780428840, -196.1311633506247745 ) ) ;
#91745=CARTESIAN_POINT ( 'NONE',  ( 35.19800885243055433, -294.7116871009865804, -258.4827826992625432 ) ) ;
#91746=CARTESIAN_POINT ( 'NONE',  ( 35.78497577281001440, -296.2662352645559167, -287.0191576251351080 ) ) ;
#91747=CARTESIAN_POINT ( 'NONE',  ( -113.4278473810832253, -295.1134496897300323, -263.9096316018108155 ) ) ;
#91748=CARTESIAN_POINT ( 'NONE',  ( -71.69384214182173309, -289.8444593454817664, -202.5683653275041252 ) ) ;
#91749=CARTESIAN_POINT ( 'NONE',  ( -93.01406652992514523, -292.6576305823376742, -222.2366695440773583 ) ) ;
#91751=CARTESIAN_POINT ( 'NONE',  ( -109.4376628559425342, -291.5225509525306506, -257.6308211104511656 ) ) ;
#91753=CARTESIAN_POINT ( 'NONE',  ( -112.9655983075335399, -291.6037549177669348, -282.5690966434786446 ) ) ;
#91754=CARTESIAN_POINT ( 'NONE',  ( 34.61279915932067297, -279.2849566659546099, -247.9790529440880391 ) ) ;
#91755=CARTESIAN_POINT ( 'NONE',  ( 33.30820374967189679, -293.3095799440126825, -251.9874661391123709 ) ) ;
#91756=CARTESIAN_POINT ( 'NONE',  ( -36.75255387050101774, -280.0593655540109808, -193.3503263514216144 ) ) ;
#91757=CARTESIAN_POINT ( 'NONE',  ( -113.7981455125467534, -284.3308724264385319, -261.4081156560843056 ) ) ;
#91758=CARTESIAN_POINT ( 'NONE',  ( 17.33345799608588322, -286.2696054494083455, -321.5314842045175396 ) ) ;
#91759=CARTESIAN_POINT ( 'NONE',  ( -101.4800478459414848, -282.1872960009666826, -307.7394249323233453 ) ) ;
#91761=CARTESIAN_POINT ( 'NONE',  ( -72.17290680989286500, -278.0798378535758388, -202.4533397644107424 ) ) ;
#91762=CARTESIAN_POINT ( 'NONE',  ( -18.24564896744194797, -285.2128513128089935, -196.0308457512828397 ) ) ;
#91764=CARTESIAN_POINT ( 'NONE',  ( -0.8789515018298554860, -294.1449983330211921, -206.1833473218507891 ) ) ;
#91765=CARTESIAN_POINT ( 'NONE',  ( 30.71718065816105181, -276.5265891308233677, -235.6250410964830451 ) ) ;
#91766=CARTESIAN_POINT ( 'NONE',  ( -36.47017944079517093, -276.7076860550151309, -343.3895319701514950 ) ) ;
#91767=CARTESIAN_POINT ( 'NONE',  ( -113.3597151247126931, -290.5655268720333879, -282.6192336813119255 ) ) ;
#91768=CARTESIAN_POINT ( 'NONE',  ( 1.335637636764364089, -280.6195446509958060, -335.2716544245148498 ) ) ;
#91769=CARTESIAN_POINT ( 'NONE',  ( 28.95660921510317820, -292.1905694134405849, -239.1296145586582043 ) ) ;
#91770=CARTESIAN_POINT ( 'NONE',  ( -102.8682676129395190, -294.0651481178776407, -306.9539161013492503 ) ) ;
#91773=CARTESIAN_POINT ( 'NONE',  ( -17.40979028262555062, -291.8239024861443340, -200.0183139752226396 ) ) ;
#91775=CARTESIAN_POINT ( 'NONE',  ( -92.08974858914540107, -281.4094976428775112, -313.9805196606274080 ) ) ;
#91776=CARTESIAN_POINT ( 'NONE',  ( -113.3670549132092873, -295.7454264841297800, -259.6376067691606409 ) ) ;
#91777=CARTESIAN_POINT ( 'NONE',  ( 19.22256250171952985, -278.9970818841499636, -219.9353566953350310 ) ) ;
#91778=CARTESIAN_POINT ( 'NONE',  ( -65.71016979450726581, -287.0039650047797863, -199.2940568747584678 ) ) ;
#91779=CARTESIAN_POINT ( 'NONE',  ( -39.97179267375241807, -285.8515069821102657, -197.4085126985433760 ) ) ;
#91780=CARTESIAN_POINT ( 'NONE',  ( -71.96295337408257353, -279.0387012991084816, -335.4297623780029198 ) ) ;
#91781=CARTESIAN_POINT ( 'NONE',  ( -109.4174155893551585, -294.8236238401540845, -250.8970348886875854 ) ) ;
#91782=CARTESIAN_POINT ( 'NONE',  ( -105.8921281902340326, -297.9435718458106521, -298.2683361158940443 ) ) ;
#91783=CARTESIAN_POINT ( 'NONE',  ( -110.6775056113343396, -277.3077303702995664, -273.3594738413528376 ) ) ;
#91786=CARTESIAN_POINT ( 'NONE',  ( -111.1963033213652068, -295.9459741385330176, -292.1157270547931262 ) ) ;
#91787=CARTESIAN_POINT ( 'NONE',  ( -107.9446695683545840, -292.7795539742988353, -246.7701259812290004 ) ) ;
#91788=CARTESIAN_POINT ( 'NONE',  ( 200.9739487937824833, 293.7020456634571701, -53.99999999999736389 ) ) ;
#91789=CARTESIAN_POINT ( 'NONE',  ( -29.15347963775107232, -289.5970591747833964, -343.0030185172483357 ) ) ;
#91792=CARTESIAN_POINT ( 'NONE',  ( -1.235477515598032872, -279.5780311815800587, -202.6177721682351205 ) ) ;
#91793=CARTESIAN_POINT ( 'NONE',  ( -112.1770765771534997, -297.4251209566139664, -252.6698992889003819 ) ) ;
#91794=CARTESIAN_POINT ( 'NONE',  ( -110.7315722883733571, -288.4517730928777155, -289.2341395093843062 ) ) ;
#91795=CARTESIAN_POINT ( 'NONE',  ( -109.8323779623486729, -297.2124640399762825, -244.4604245824954205 ) ) ;
#91796=CARTESIAN_POINT ( 'NONE',  ( 35.66326375148873495, -293.9266412847684364, -273.4856438674964920 ) ) ;
#91800=CARTESIAN_POINT ( 'NONE',  ( 22.75351225982018732, -289.7066959741308665, -317.4063404058811102 ) ) ;
#91801=CARTESIAN_POINT ( 'NONE',  ( -72.02372285203398405, -279.9805209788415823, -342.4524372437778652 ) ) ;
#91802=CARTESIAN_POINT ( 'NONE',  ( 37.76417643443183891, -281.1081970956980172, -286.9270524464232608 ) ) ;
#91803=CARTESIAN_POINT ( 'NONE',  ( -109.1205617816469129, -286.8275520536594740, -249.0193444161533591 ) ) ;
#91804=CARTESIAN_POINT ( 'NONE',  ( -5.006668005434542046, -285.0443140911882551, -201.1292467610936967 ) ) ;
#91805=CARTESIAN_POINT ( 'NONE',  ( -92.45595725158084122, -271.2609296138390960, -219.7215374228372013 ) ) ;
#91806=CARTESIAN_POINT ( 'NONE',  ( -43.62762957097055505, -275.8924144356403190, -196.1352781762911945 ) ) ;
#91807=CARTESIAN_POINT ( 'NONE',  ( -109.4983884083058854, -288.8694035462945635, -252.0138120648957454 ) ) ;
#91808=CARTESIAN_POINT ( 'NONE',  ( -88.36255563599863194, -279.6185667387573517, -326.3716329020712692 ) ) ;
#91810=CARTESIAN_POINT ( 'NONE',  ( -76.82185668607338869, -279.5076366028725943, -208.8979501364676707 ) ) ;
#91811=CARTESIAN_POINT ( 'NONE',  ( -27.53650123667327776, -279.5284492524394295, -197.8684942311847124 ) ) ;
#91812=CARTESIAN_POINT ( 'NONE',  ( 37.29423665495373541, -276.8539013933267370, -288.0520528909956397 ) ) ;
#91813=CARTESIAN_POINT ( 'NONE',  ( -74.80030153582180219, -278.3597924952936182, -203.5414958685116460 ) ) ;
#91814=CARTESIAN_POINT ( 'NONE',  ( 4.282212335244459211, -58.25047808272906025, -351.9149493628895584 ) ) ;
#91815=CARTESIAN_POINT ( 'NONE',  ( -18.61899987255275946, -275.2287030145972722, -195.8597626330902983 ) ) ;
#91816=CARTESIAN_POINT ( 'NONE',  ( -51.70776717304013914, -299.2972395592836961, -195.2590580967229812 ) ) ;
#91817=CARTESIAN_POINT ( 'NONE',  ( 10.59707575819634329, -289.1948066931273615, -210.1954327657594490 ) ) ;
#91819=CARTESIAN_POINT ( 'NONE',  ( 35.30053514148841032, -288.4973683995830811, -260.1251577783254447 ) ) ;
#91820=CARTESIAN_POINT ( 'NONE',  ( 19.82553354330629602, -289.9987018940424832, -320.4395068173125765 ) ) ;
#91821=CARTESIAN_POINT ( 'NONE',  ( -105.8031890486252991, -290.2439073460990926, -244.5871305292801026 ) ) ;
#91822=CARTESIAN_POINT ( 'NONE',  ( -90.40024388924976506, -283.2865065463062706, -326.1505799899610452 ) ) ;
#91823=CARTESIAN_POINT ( 'NONE',  ( 20.31364087874701951, -279.3082717431319679, -224.2926681367810602 ) ) ;
#91824=CARTESIAN_POINT ( 'NONE',  ( -80.03876101613434457, -287.3283573091060816, -209.5705195250062616 ) ) ;
#91825=CARTESIAN_POINT ( 'NONE',  ( 32.88619890473360385, -280.3273064246847639, -292.8598822282093579 ) ) ;
#91826=CARTESIAN_POINT ( 'NONE',  ( -57.26286389490530837, -281.1048254673006568, -199.6193996619407756 ) ) ;
#91827=CARTESIAN_POINT ( 'NONE',  ( -53.96184027778807035, -277.7635378514856939, -341.5593444223308097 ) ) ;
#91828=CARTESIAN_POINT ( 'NONE',  ( -112.9704871889050963, -289.1939925663604072, -282.5387731981658703 ) ) ;
#91829=CARTESIAN_POINT ( 'NONE',  ( -97.04045901947404218, -284.7045630008437911, -318.7575810530527747 ) ) ;
#91830=CARTESIAN_POINT ( 'NONE',  ( -55.68143276528162744, -283.7744671459013830, -345.0818052776580771 ) ) ;
#91831=CARTESIAN_POINT ( 'NONE',  ( 31.97593600518977652, -281.4130346249777404, -247.3093392063195211 ) ) ;
#91834=CARTESIAN_POINT ( 'NONE',  ( -71.63472046504641355, -293.4644308327153226, -202.7871904682546358 ) ) ;
#91835=CARTESIAN_POINT ( 'NONE',  ( -64.19989079931440301, -290.3939113357287169, -198.6677790883814509 ) ) ;
#91836=CARTESIAN_POINT ( 'NONE',  ( 35.07612058973654001, -274.4663030009210161, -259.3648356892419997 ) ) ;
#91838=CARTESIAN_POINT ( 'NONE',  ( -105.8706357552103299, -295.4495753946923173, -305.3653693011394239 ) ) ;
#91839=CARTESIAN_POINT ( 'NONE',  ( -19.88936985730601137, -290.7603060234929444, -198.7113942926003460 ) ) ;
#91840=CARTESIAN_POINT ( 'NONE',  ( 23.75700681572322637, -292.3663860301136310, -312.2229679927377219 ) ) ;
#91841=CARTESIAN_POINT ( 'NONE',  ( -73.72855007748313483, -290.7517836848141997, -334.1182738369247431 ) ) ;
#91842=CARTESIAN_POINT ( 'NONE',  ( 133.0380396672494783, -299.5541904835127980, -189.2093064027359901 ) ) ;
#91843=CARTESIAN_POINT ( 'NONE',  ( -110.3756761777892734, -292.7713613656292750, -253.3012529244568327 ) ) ;
#91844=CARTESIAN_POINT ( 'NONE',  ( 37.40593867008024631, -291.4443189539040304, -261.9568209886302270 ) ) ;
#91845=CARTESIAN_POINT ( 'NONE',  ( 21.89687321264483089, -296.1831772298917826, -316.3793056893565563 ) ) ;
#91846=CARTESIAN_POINT ( 'NONE',  ( -52.14817795662543887, -286.7991715726088842, -198.6382021069378254 ) ) ;
#91847=CARTESIAN_POINT ( 'NONE',  ( 25.00566051432071291, -296.1189489545133711, -312.3472472124772139 ) ) ;
#91849=CARTESIAN_POINT ( 'NONE',  ( 38.06180751901270298, -277.5418625123454035, -271.1291655900909632 ) ) ;
#91850=CARTESIAN_POINT ( 'NONE',  ( -112.9665071198076021, -272.0788151381000830, -256.1413742479614939 ) ) ;
#91851=CARTESIAN_POINT ( 'NONE',  ( 36.36107723001683922, -273.8801293882200412, -277.1341986536174886 ) ) ;
#91852=CARTESIAN_POINT ( 'NONE',  ( 8.039176767074440733, -278.7573703702663011, -211.2883394012095266 ) ) ;
#91853=CARTESIAN_POINT ( 'NONE',  ( -74.48751654362214936, -274.7516660076539665, -206.9988494864960558 ) ) ;
#91855=CARTESIAN_POINT ( 'NONE',  ( -100.6643184575767265, -297.4651814447006473, -307.9530244787657125 ) ) ;
#91857=CARTESIAN_POINT ( 'NONE',  ( -100.3002295447359273, -296.8428419755931600, -307.7277943024036517 ) ) ;
#91858=DIRECTION ( 'NONE',  ( 0.000000000000000000, 0.000000000000000000, 1.000000000000000000 ) ) ;
#91859=CARTESIAN_POINT ( 'NONE',  ( 37.93604199813501054, -285.5157656970316680, -265.9405660656128703 ) ) ;
#91860=CARTESIAN_POINT ( 'NONE',  ( -69.48904837939930701, -273.4501191088235146, -204.8206876746464218 ) ) ;
#91861=CARTESIAN_POINT ( 'NONE',  ( 1.521678898389058121, -286.5565626252717948, -203.8729447923337545 ) ) ;
#91862=CARTESIAN_POINT ( 'NONE',  ( -68.04934297520905773, -289.1111759990607766, -340.9499624437111720 ) ) ;
#91863=CARTESIAN_POINT ( 'NONE',  ( -109.9992654286719613, -298.2762687694247461, -290.3432352252511350 ) ) ;
#91864=CARTESIAN_POINT ( 'NONE',  ( -58.96164863047513194, -293.3323655883094148, -342.0033279630837342 ) ) ;
#91865=CARTESIAN_POINT ( 'NONE',  ( 37.17715946099330893, -280.5143881901126974, -251.6234984260304941 ) ) ;
#91866=CARTESIAN_POINT ( 'NONE',  ( -95.99890600148557951, -293.4094976428775681, -317.0979686699210447 ) ) ;
#91867=CARTESIAN_POINT ( 'NONE',  ( -101.8277212569831391, -277.0654772562059520, -231.9657784740427360 ) ) ;
#91868=CARTESIAN_POINT ( 'NONE',  ( -95.27339438497588731, -288.7153551414180015, -315.4485938646981822 ) ) ;
#91870=CARTESIAN_POINT ( 'NONE',  ( -93.93726597655496846, -287.8683913119828048, -319.6519974895999212 ) ) ;
#91871=CARTESIAN_POINT ( 'NONE',  ( -33.78388818234863322, -299.6975443180613183, -196.5601236198808408 ) ) ;
#91872=CARTESIAN_POINT ( 'NONE',  ( 35.60773147979883646, -282.6895716546461017, -247.6237759881351792 ) ) ;
#91873=CARTESIAN_POINT ( 'NONE',  ( -106.7449695285716018, -271.0213444609829025, -240.3541517011892665 ) ) ;
#91874=CARTESIAN_POINT ( 'NONE',  ( 35.68737416741759461, -281.5287034445308905, -268.5835766000296871 ) ) ;
#91875=CARTESIAN_POINT ( 'NONE',  ( -95.57249168267412642, -297.4000665056227035, -219.9012354232556277 ) ) ;
#91876=CARTESIAN_POINT ( 'NONE',  ( -90.63575263835306828, -274.7035018539475004, -219.5970478485548369 ) ) ;
#91877=CARTESIAN_POINT ( 'NONE',  ( 37.91106703316073379, -285.7187508110668546, -277.1681166480832417 ) ) ;
#91878=CARTESIAN_POINT ( 'NONE',  ( -39.55445629143974884, -282.0245547042659382, -195.3810513015654067 ) ) ;
#91879=CARTESIAN_POINT ( 'NONE',  ( -63.40381652690489744, -272.6247474751405662, -201.8275555931272152 ) ) ;
#91882=CARTESIAN_POINT ( 'NONE',  ( -77.96487866844292114, -287.4836577092515881, -207.6770657199440393 ) ) ;
#91884=CARTESIAN_POINT ( 'NONE',  ( 13.84574458161073807, -272.1952119285918457, -206.2264541496106460 ) ) ;
#91885=CARTESIAN_POINT ( 'NONE',  ( 21.60017092007287687, -275.4141205316000764, -319.6562968383907446 ) ) ;
#91886=CARTESIAN_POINT ( 'NONE',  ( -91.23543323702172358, -285.3562470314963093, -320.6221693475289953 ) ) ;
#91887=CARTESIAN_POINT ( 'NONE',  ( 21.30499631019853268, -276.5288173438711397, -225.5407098235782826 ) ) ;
#91888=CARTESIAN_POINT ( 'NONE',  ( -110.5382745982274173, -285.6995892137407509, -292.3352137674459073 ) ) ;
#91889=CARTESIAN_POINT ( 'NONE',  ( -56.43690790025585358, -282.0987019870414656, -341.2307415448175902 ) ) ;
#91890=CARTESIAN_POINT ( 'NONE',  ( 34.64734469879528689, -283.2814240066580851, -249.3235783220800386 ) ) ;
#91891=CARTESIAN_POINT ( 'NONE',  ( -41.19489415316546399, -274.1717271464443115, -193.4053284942501136 ) ) ;
#91892=CARTESIAN_POINT ( 'NONE',  ( 38.92446846478642897, -275.2528393179302952, -259.7558583125066889 ) ) ;
#91893=CARTESIAN_POINT ( 'NONE',  ( -45.21928212433525118, -297.0727189644497912, -344.4345994803593953 ) ) ;
#91896=CARTESIAN_POINT ( 'NONE',  ( -78.82085296595143120, -293.7443424706657993, -333.7628952348099460 ) ) ;
#91898=CARTESIAN_POINT ( 'NONE',  ( -11.23790622253789984, -276.2102227427271828, -338.6002591364451746 ) ) ;
#91899=CARTESIAN_POINT ( 'NONE',  ( -113.9446275073758699, -273.7570339554058592, -270.3764274833388868 ) ) ;
#91900=CARTESIAN_POINT ( 'NONE',  ( -74.07780344596864097, -287.3170995385450510, -206.0935373704038795 ) ) ;
#91901=CARTESIAN_POINT ( 'NONE',  ( 15.01713785587491401, -295.8495755538914409, -325.8702148620531034 ) ) ;
#91902=CARTESIAN_POINT ( 'NONE',  ( 15.21745189415454114, -295.5345800671756251, -326.0885282622135151 ) ) ;
#91903=CARTESIAN_POINT ( 'NONE',  ( -73.53544701219848889, -293.5712964389833246, -204.8044734432176313 ) ) ;
#91904=CARTESIAN_POINT ( 'NONE',  ( -43.88667278441708675, -277.9692035606976788, -195.7630480247708249 ) ) ;
#91905=CARTESIAN_POINT ( 'NONE',  ( -67.91972832504953317, -281.5677790049043665, -202.4775244486798158 ) ) ;
#91906=CARTESIAN_POINT ( 'NONE',  ( -110.0026929880996249, -294.4227261725366702, -286.5380867493872756 ) ) ;
#91907=CARTESIAN_POINT ( 'NONE',  ( -4.674599227087804287, -284.4868630699195364, -338.7359360913204682 ) ) ;
#91908=CARTESIAN_POINT ( 'NONE',  ( -52.13794709388877635, -284.7785734099470005, -198.5607200144326612 ) ) ;
#91909=CARTESIAN_POINT ( 'NONE',  ( 201.4154447744461436, 287.2677491621798254, -97.13488168232527187 ) ) ;
#91911=CARTESIAN_POINT ( 'NONE',  ( -54.75726958385478582, -285.4889231387453492, -199.3948759657450864 ) ) ;
#91913=CARTESIAN_POINT ( 'NONE',  ( 38.12387407597498168, -282.8041900982574930, -284.0884207088452627 ) ) ;
#91914=CARTESIAN_POINT ( 'NONE',  ( -62.04083777113134346, -274.0552430078333828, -201.6440161341498083 ) ) ;
#91915=CARTESIAN_POINT ( 'NONE',  ( 35.47640323013938257, -286.0444184606371891, -246.4104449699778172 ) ) ;
#91916=CARTESIAN_POINT ( 'NONE',  ( -111.2108243040277102, -279.2308470294760241, -291.2458661682531442 ) ) ;
#91917=CARTESIAN_POINT ( 'NONE',  ( -109.0782685117798820, -279.7389951790068494, -296.5265881705340121 ) ) ;
#91918=CARTESIAN_POINT ( 'NONE',  ( 19.07972590216577657, -281.4908782539976642, -218.1123335820869045 ) ) ;
#91919=CARTESIAN_POINT ( 'NONE',  ( -102.0172624299487154, -276.4809262143062369, -239.1787733560258289 ) ) ;
#91920=CARTESIAN_POINT ( 'NONE',  ( 168.9861705969244952, 232.0887483361810553, -192.7465431548272932 ) ) ;
#91922=CARTESIAN_POINT ( 'NONE',  ( 8.432731809881056861, -276.6807212603808352, -211.1603595064202068 ) ) ;
#91923=CARTESIAN_POINT ( 'NONE',  ( 160.6459981038951241, 220.5539213599568882, -205.1006532850495319 ) ) ;
#91924=CARTESIAN_POINT ( 'NONE',  ( -110.2069566012316244, -276.7819686512834210, -254.1008076556053368 ) ) ;
#91925=CARTESIAN_POINT ( 'NONE',  ( 33.50974497670642194, -294.9581110484263036, -242.7559094410300702 ) ) ;
#91926=CARTESIAN_POINT ( 'NONE',  ( -12.98208472004965763, -294.0757943326610757, -339.3383318844054202 ) ) ;
#91927=CARTESIAN_POINT ( 'NONE',  ( -60.01512694401825598, -288.8459964239874012, -343.8828332748200864 ) ) ;
#91929=CARTESIAN_POINT ( 'NONE',  ( -70.56818840286992156, -294.0563422331115930, -339.1839972827448833 ) ) ;
#91930=CARTESIAN_POINT ( 'NONE',  ( -42.71223244418801812, -284.3831666969355751, -196.7440212856437540 ) ) ;
#91931=CARTESIAN_POINT ( 'NONE',  ( -67.08028788448426383, -293.5185224848062830, -202.3428713081064245 ) ) ;
#91932=CARTESIAN_POINT ( 'NONE',  ( 11.60892536227643923, -285.2256131238391959, -215.2058446102657285 ) ) ;
#91933=CARTESIAN_POINT ( 'NONE',  ( -93.64361965568940604, -286.5336010592957905, -223.1240844515426147 ) ) ;
#91935=CARTESIAN_POINT ( 'NONE',  ( -99.02270762608848997, -292.1029866440836145, -224.6414619417408005 ) ) ;
#91936=CARTESIAN_POINT ( 'NONE',  ( 34.29225727024859083, -282.2347667020269455, -284.7964595700007635 ) ) ;
#91937=CARTESIAN_POINT ( 'NONE',  ( -111.2131959168634694, -295.0918155158527725, -290.6345199974070965 ) ) ;
#91938=CARTESIAN_POINT ( 'NONE',  ( -113.9506063685677333, -291.2724074518176849, -276.9499439747928591 ) ) ;
#91939=CARTESIAN_POINT ( 'NONE',  ( -112.2013555857373746, -290.8214502075636005, -288.1814473201278588 ) ) ;
#91940=CARTESIAN_POINT ( 'NONE',  ( 12.15736005180612800, -288.5073287863922360, -324.0846597465782111 ) ) ;
#91943=CARTESIAN_POINT ( 'NONE',  ( -112.7120078377118233, -298.3144246460426530, -278.0826589455841145 ) ) ;
#91944=CARTESIAN_POINT ( 'NONE',  ( -51.69158880102221332, -296.5572342895215456, -195.1580839439134820 ) ) ;
#91945=CARTESIAN_POINT ( 'NONE',  ( -11.64940865082109411, -279.4537228864278404, -201.7267683024158487 ) ) ;
#91948=CARTESIAN_POINT ( 'NONE',  ( 37.57642738403805538, -274.8399216343725016, -252.7880495320005707 ) ) ;
#91949=CARTESIAN_POINT ( 'NONE',  ( -96.64687811334589185, -295.6396275759994410, -226.5950656291205405 ) ) ;
#91950=CARTESIAN_POINT ( 'NONE',  ( -35.05626805444299521, -278.8835642863836028, -344.5611333663245546 ) ) ;
#91951=CARTESIAN_POINT ( 'NONE',  ( 28.97518455151838168, -273.2465126446829800, -237.0004182916892432 ) ) ;
#91952=CARTESIAN_POINT ( 'NONE',  ( -90.68532492310458792, -297.0342764166445590, -320.8484608131063283 ) ) ;
#91953=CARTESIAN_POINT ( 'NONE',  ( -34.27455773902066483, -296.0923594263009022, -343.6060407542240114 ) ) ;
#91955=CARTESIAN_POINT ( 'NONE',  ( -55.85598205364291147, -296.8868124432819968, -344.2777046070123106 ) ) ;
#91956=CARTESIAN_POINT ( 'NONE',  ( -64.84684375226086672, -295.6937435332915243, -200.3519702175213979 ) ) ;
#91957=CARTESIAN_POINT ( 'NONE',  ( -3.596568554813896590, -293.1613592672813979, -205.5139224875146056 ) ) ;
#91958=CARTESIAN_POINT ( 'NONE',  ( 1.105749626554779264, -275.3545969431295362, -203.8180340006146594 ) ) ;
#91959=CARTESIAN_POINT ( 'NONE',  ( -100.2056147587211541, -289.6495546316100445, -232.1053582376200666 ) ) ;
#91961=CARTESIAN_POINT ( 'NONE',  ( -92.12964482789575982, -273.7870400243897393, -216.3443796625153084 ) ) ;
#91962=CARTESIAN_POINT ( 'NONE',  ( -109.1621552512183797, -296.7106070021491746, -283.6178463856912799 ) ) ;
#91963=CARTESIAN_POINT ( 'NONE',  ( -45.12901951119007293, -281.9340233236259223, -195.3575115912544220 ) ) ;
#91964=CARTESIAN_POINT ( 'NONE',  ( 39.14832307778954856, -280.1958719896468892, -267.0952412762640620 ) ) ;
#91965=CARTESIAN_POINT ( 'NONE',  ( -84.80998275992679680, -277.0354545267573485, -330.9273373640988325 ) ) ;
#91966=CARTESIAN_POINT ( 'NONE',  ( -6.534919710642594026, -278.8498476236773627, -200.6520660626392782 ) ) ;
#91967=CARTESIAN_POINT ( 'NONE',  ( 30.38103407202071082, -279.1220303900754516, -237.6274914876550497 ) ) ;
#91969=CARTESIAN_POINT ( 'NONE',  ( 15.88543004276931825, -273.3990933848373288, -219.4715144374321483 ) ) ;
#91970=CARTESIAN_POINT ( 'NONE',  ( -88.12214496503453631, -279.7625257247373725, -325.6245846552706098 ) ) ;
#91973=FACE_OUTER_BOUND ( 'NONE', #43521, .T. ) ;
#91974=CARTESIAN_POINT ( 'NONE',  ( -40.37703197663353194, -296.2544867127755310, -194.3836547306584919 ) ) ;
#91975=CARTESIAN_POINT ( 'NONE',  ( -36.37836834806066122, -292.0639173955225374, -193.3541118592440000 ) ) ;
#91977=CARTESIAN_POINT ( 'NONE',  ( 21.22887725293852768, -278.1992681506508802, -317.4932249393975212 ) ) ;
#91978=CARTESIAN_POINT ( 'NONE',  ( 14.90774451288066693, -272.7886193610837609, -216.5559492543085014 ) ) ;
#91980=CARTESIAN_POINT ( 'NONE',  ( -3.515140457016934672, -284.5293911776420828, -337.9408604897415103 ) ) ;
#91982=CARTESIAN_POINT ( 'NONE',  ( 7.768505764125121615, -284.6675049210330712, -210.3796399163485091 ) ) ;
#91984=CARTESIAN_POINT ( 'NONE',  ( -23.45868950761676786, -293.6657704200166563, -342.4851353964479017 ) ) ;
#91985=CARTESIAN_POINT ( 'NONE',  ( 26.75072558276606927, -286.1985290916646818, -307.9196834629384512 ) ) ;
#91987=CARTESIAN_POINT ( 'NONE',  ( 28.91325046412860189, -292.0193218077198480, -305.6186068693261859 ) ) ;
#91988=CARTESIAN_POINT ( 'NONE',  ( -21.11238584718955380, -284.7366129088260891, -195.8002897356844301 ) ) ;
#91989=CARTESIAN_POINT ( 'NONE',  ( -88.09543143389169018, -280.9281100523474493, -216.7134359059565725 ) ) ;
#91990=CARTESIAN_POINT ( 'NONE',  ( 38.57968083735106291, -288.6290522371708107, -260.1654016927717521 ) ) ;
#91991=CARTESIAN_POINT ( 'NONE',  ( 32.25394314418228703, -279.3978389811244938, -239.8583238657862751 ) ) ;
#91992=CARTESIAN_POINT ( 'NONE',  ( 34.75922159645808307, -287.7038752945713327, -281.8625601182478704 ) ) ;
#91993=CARTESIAN_POINT ( 'NONE',  ( -39.73846186487903509, -281.4467730477243776, -196.7983073072052775 ) ) ;
#91994=CARTESIAN_POINT ( 'NONE',  ( 23.81189559993686800, -281.7983218556843212, -230.1096022833589529 ) ) ;
#91995=CARTESIAN_POINT ( 'NONE',  ( 8.783644447499016295, -288.6609627192716516, -210.7720301598189394 ) ) ;
#91997=CARTESIAN_POINT ( 'NONE',  ( -75.77806400934161957, -297.3875275589903140, -203.5792702333208126 ) ) ;
#91998=CARTESIAN_POINT ( 'NONE',  ( -111.9814579140253556, -292.5208526317213682, -271.2290795190710924 ) ) ;
#92000=CARTESIAN_POINT ( 'NONE',  ( -88.52914483777347243, -299.9090924074130271, -206.2264541496106460 ) ) ;
#92001=VERTEX_POINT ( 'NONE', #51975 ) ;
#92002=CARTESIAN_POINT ( 'NONE',  ( -68.07070580768768764, -271.6494982618768859, -201.7485503678572343 ) ) ;
#92004=CARTESIAN_POINT ( 'NONE',  ( -110.8259917662915370, -294.6968267037566420, -290.5229457555069530 ) ) ;
#92005=CARTESIAN_POINT ( 'NONE',  ( 51.77000390654524864, -298.7049638229934203, -197.3073222814579708 ) ) ;
#92006=CARTESIAN_POINT ( 'NONE',  ( -73.87198977184749538, -291.0667790645606487, -334.3775839084418635 ) ) ;
#92008=CARTESIAN_POINT ( 'NONE',  ( 36.44112851301330380, -283.3963049185937848, -276.8175352054258838 ) ) ;
#92009=CARTESIAN_POINT ( 'NONE',  ( -110.9693100189715125, -291.7194235732703760, -290.7959254338969117 ) ) ;
#92010=CARTESIAN_POINT ( 'NONE',  ( -99.46000844568962407, -291.2712631964897128, -315.0446589745617416 ) ) ;
#92011=CARTESIAN_POINT ( 'NONE',  ( -69.65919759463426431, -287.6268861137378394, -202.6669655641330507 ) ) ;
#92012=CARTESIAN_POINT ( 'NONE',  ( -16.99403352886174190, -280.4745445257507868, -196.0982573559109881 ) ) ;
#92013=CARTESIAN_POINT ( 'NONE',  ( -110.2099275173082020, -294.3768527458136646, -290.3495055397546025 ) ) ;
#92014=CARTESIAN_POINT ( 'NONE',  ( 25.10604466883235020, -281.9830244842723914, -315.4310201944050505 ) ) ;
#92015=CARTESIAN_POINT ( 'NONE',  ( 34.70229330404547596, -277.1802454070192994, -252.4578084109721487 ) ) ;
#92016=CARTESIAN_POINT ( 'NONE',  ( -110.4683760289727132, -299.2662352645559167, -253.7030783399848985 ) ) ;
#92017=CARTESIAN_POINT ( 'NONE',  ( 36.95933304926105478, -273.5895259923603362, -254.3831637393510050 ) ) ;
#92019=CARTESIAN_POINT ( 'NONE',  ( 33.99914805675263807, -281.2675685681434743, -286.1241069803528490 ) ) ;
#92020=CARTESIAN_POINT ( 'NONE',  ( -111.7856387412321197, -279.5295139327766378, -288.4744952184310591 ) ) ;
#92021=CARTESIAN_POINT ( 'NONE',  ( -103.8306470437137534, -284.1124130479129235, -231.8882622163514782 ) ) ;
#92022=CARTESIAN_POINT ( 'NONE',  ( -41.67426004594123867, -293.7571183094771641, -196.4241610917527510 ) ) ;
#92023=CARTESIAN_POINT ( 'NONE',  ( -87.52499333443032015, -274.9659601317374040, -212.9491883737881039 ) ) ;
#92024=CARTESIAN_POINT ( 'NONE',  ( -99.17842488240971477, -274.4700719676970380, -225.2230780620052712 ) ) ;
#92026=CARTESIAN_POINT ( 'NONE',  ( 33.89279848684195429, -275.5967291786685678, -286.3755898579345853 ) ) ;
#92027=CARTESIAN_POINT ( 'NONE',  ( -94.46578244691021098, -297.8818750915947930, -318.7221195585580062 ) ) ;
#92028=CARTESIAN_POINT ( 'NONE',  ( -40.01451821524881325, -284.0183229289527844, -195.5755279760670078 ) ) ;
#92029=CARTESIAN_POINT ( 'NONE',  ( 39.58559932006338755, -293.2541105181479111, -273.1780118490173095 ) ) ;
#92030=CARTESIAN_POINT ( 'NONE',  ( 33.63344882615579223, -273.2703432677488991, -247.0781140317762947 ) ) ;
#92031=CARTESIAN_POINT ( 'NONE',  ( 34.32707485210553955, -289.4843486069773917, -296.3996331080620621 ) ) ;
#92032=CARTESIAN_POINT ( 'NONE',  ( -110.0979748727744720, -289.3544335453830740, -279.3472494500714447 ) ) ;
#92034=CARTESIAN_POINT ( 'NONE',  ( -8.714997057639369160, -290.9942222789335915, -199.5153830048110422 ) ) ;
#92035=CARTESIAN_POINT ( 'NONE',  ( -110.2665035933152780, -290.2799426631613073, -265.7300492090016064 ) ) ;
#92037=CARTESIAN_POINT ( 'NONE',  ( 23.60736984058561916, -288.0084566337292244, -223.7917301608247556 ) ) ;
#92038=CARTESIAN_POINT ( 'NONE',  ( -89.49165153032868147, -279.6257366972444061, -219.1771265859307505 ) ) ;
#92040=CARTESIAN_POINT ( 'NONE',  ( -94.43070419324349984, -294.7747330633922616, -321.5894578174184062 ) ) ;
#92041=CARTESIAN_POINT ( 'NONE',  ( -12.74417551216628652, -287.0151327517111781, -197.5032112793357157 ) ) ;
#92042=CARTESIAN_POINT ( 'NONE',  ( -43.66876323159878126, -286.3076894294931662, -193.5894754655832912 ) ) ;
#92044=CARTESIAN_POINT ( 'NONE',  ( -37.53631795842395746, -283.3879720882690094, -343.3944356157275593 ) ) ;
#92045=CARTESIAN_POINT ( 'NONE',  ( -104.3679765323354616, -256.1617121061207740, -326.7344306583073035 ) ) ;
#92046=CARTESIAN_POINT ( 'NONE',  ( 4.264052385521533317, -57.87785853924207657, -353.4280301830093549 ) ) ;
#92047=CARTESIAN_POINT ( 'NONE',  ( 166.5363578158908240, 230.4628405918484475, -189.9770653364864472 ) ) ;
#92048=CARTESIAN_POINT ( 'NONE',  ( 34.32067219484060416, -274.9432610931079353, -285.0956393696828286 ) ) ;
#92049=CARTESIAN_POINT ( 'NONE',  ( 24.05988102136718254, -273.9198550864552431, -230.3102515012598133 ) ) ;
#92050=CARTESIAN_POINT ( 'NONE',  ( -112.2130229303147928, -296.2815456867034527, -252.6463804626246201 ) ) ;
#92051=CARTESIAN_POINT ( 'NONE',  ( -92.95586860365406778, -239.4756788387215352, -338.8937605817495751 ) ) ;
#92052=CARTESIAN_POINT ( 'NONE',  ( 12.37139436456461716, -275.0612863531230801, -328.5152795485695947 ) ) ;
#92053=CARTESIAN_POINT ( 'NONE',  ( -92.79201071169505610, -275.0030598458685063, -221.3382960424069097 ) ) ;
#92054=CARTESIAN_POINT ( 'NONE',  ( -49.75453633662386466, -292.9699190552871642, -198.0589850946062995 ) ) ;
#92056=CARTESIAN_POINT ( 'NONE',  ( -113.5426695157466952, -297.6098935921430666, -261.0749736215325356 ) ) ;
#92057=CARTESIAN_POINT ( 'NONE',  ( 35.61368441934300222, -287.9814376395827935, -265.5764307693015098 ) ) ;
#92058=CARTESIAN_POINT ( 'NONE',  ( -33.43280527484429143, -295.8069798995209680, -347.1132439189937031 ) ) ;
#92059=CARTESIAN_POINT ( 'NONE',  ( -90.66490207147944602, -296.2757623633210642, -325.8976296311550982 ) ) ;
#92060=CARTESIAN_POINT ( 'NONE',  ( 32.62846924756416200, -293.4413093988539458, -249.3740805853048812 ) ) ;
#92061=VERTEX_POINT ( 'NONE', #43935 ) ;
#92062=CARTESIAN_POINT ( 'NONE',  ( 37.06964831873957422, -277.3040884406809141, -257.1623273905797760 ) ) ;
#92064=CARTESIAN_POINT ( 'NONE',  ( -50.92260395706821896, -279.3907192836596778, -194.6307676977707501 ) ) ;
#92066=CARTESIAN_POINT ( 'NONE',  ( -92.89733007106960372, -278.8161941620347761, -318.0788340878128224 ) ) ;
#92067=CARTESIAN_POINT ( 'NONE',  ( -16.08263755026676023, -276.0833610950304546, -197.3542936509817025 ) ) ;
#92068=CARTESIAN_POINT ( 'NONE',  ( -111.4526897081685206, -276.3970826590530692, -284.0691491544161522 ) ) ;
#92069=CARTESIAN_POINT ( 'NONE',  ( -109.1473611472535765, -297.3849921027006076, -256.5889477398108625 ) ) ;
#92070=CARTESIAN_POINT ( 'NONE',  ( -109.1709386364213543, -294.9175278265370821, -286.3590995554434926 ) ) ;
#92072=CARTESIAN_POINT ( 'NONE',  ( -42.43224750726681549, -280.4819101112354360, -193.5912460883368738 ) ) ;
#92073=CARTESIAN_POINT ( 'NONE',  ( 25.37665491622757230, -276.2324032763314676, -307.7162775328546331 ) ) ;
#92074=CARTESIAN_POINT ( 'NONE',  ( 4.921299900166357766, -285.2947579352629646, -206.5238996140087124 ) ) ;
#92075=CARTESIAN_POINT ( 'NONE',  ( -84.09644513435723923, -299.4112751574487561, -211.5051731440177321 ) ) ;
#92076=CARTESIAN_POINT ( 'NONE',  ( 82.62096999362312033, -301.7479467211907149, -196.5710693965175437 ) ) ;
#92077=CARTESIAN_POINT ( 'NONE',  ( 31.54801855125912624, -287.0765860671094174, -294.9945990004187593 ) ) ;
#92078=CARTESIAN_POINT ( 'NONE',  ( -79.61554045679248759, -277.7119601983326902, -209.6083696056004442 ) ) ;
#92079=CARTESIAN_POINT ( 'NONE',  ( -11.51952119948420439, -278.9697806391696986, -201.3972093027971937 ) ) ;
#92080=CARTESIAN_POINT ( 'NONE',  ( -110.3973360645508421, -282.4471423871152638, -284.6505636823185341 ) ) ;
#92081=CARTESIAN_POINT ( 'NONE',  ( -10.34543797468004911, -288.4045760319200440, -200.3745887515610775 ) ) ;
#92082=CARTESIAN_POINT ( 'NONE',  ( -83.24319208077670851, -278.9018947472122250, -327.6994059298249340 ) ) ;
#92084=CARTESIAN_POINT ( 'NONE',  ( -17.18914787079680906, -294.3124661108431610, -198.1193344808359029 ) ) ;
#92085=CARTESIAN_POINT ( 'NONE',  ( -98.00811692064213787, -276.1743449035008666, -316.1379165729312604 ) ) ;
#92086=CARTESIAN_POINT ( 'NONE',  ( -56.61907550713243609, -277.9585795022109096, -340.9280509072449377 ) ) ;
#92087=CARTESIAN_POINT ( 'NONE',  ( 23.63533713568915928, -284.1495149366861028, -314.3355571250510820 ) ) ;
#92089=CARTESIAN_POINT ( 'NONE',  ( -38.86614059597783211, -290.9912866863014642, -345.9057424287087201 ) ) ;
#92090=CARTESIAN_POINT ( 'NONE',  ( -111.1827526396086796, -294.3824330138968435, -283.5667972832322903 ) ) ;
#92093=CARTESIAN_POINT ( 'NONE',  ( 3.215954506125094259, -273.2941128010002103, -209.0114635707370496 ) ) ;
#92094=CARTESIAN_POINT ( 'NONE',  ( 15.77561970220103404, -290.9532700453690950, -218.4278891622215326 ) ) ;
#92097=CARTESIAN_POINT ( 'NONE',  ( -90.29077295507200063, -289.7996606162673174, -215.3414338584399843 ) ) ;
#92098=CARTESIAN_POINT ( 'NONE',  ( -94.89624433596443964, -285.5063151616044479, -316.5755298017816131 ) ) ;
#92099=CARTESIAN_POINT ( 'NONE',  ( 17.63406156653762480, -285.0644993850514197, -217.8291359498942086 ) ) ;
#92100=CARTESIAN_POINT ( 'NONE',  ( -108.6598237742127537, -285.7399014278877871, -288.5022358712301980 ) ) ;
#92102=CARTESIAN_POINT ( 'NONE',  ( -74.81157098468700895, -286.3422261880000974, -207.5231477339215758 ) ) ;
#92103=CARTESIAN_POINT ( 'NONE',  ( -110.4061193128121943, -292.7683902754417886, -251.8700526055010016 ) ) ;
#92105=CARTESIAN_POINT ( 'NONE',  ( 38.18290392137456735, -273.6783662369252852, -273.9994752100878372 ) ) ;
#92106=CARTESIAN_POINT ( 'NONE',  ( 32.53208464009873069, -275.4706213075840537, -237.9325165720736948 ) ) ;
#92107=CARTESIAN_POINT ( 'NONE',  ( -108.5175170296699463, -288.3039852311906657, -295.8800774431864511 ) ) ;
#92108=CARTESIAN_POINT ( 'NONE',  ( -69.01537505253617155, -277.4572722322339473, -340.5594118909148165 ) ) ;
#92109=CARTESIAN_POINT ( 'NONE',  ( -85.52092927726266680, -297.7017159697305146, -327.4430724511720427 ) ) ;
#92112=CARTESIAN_POINT ( 'NONE',  ( -101.4130973739320893, -283.7275272302651388, -234.2554835568423073 ) ) ;
#92113=CARTESIAN_POINT ( 'NONE',  ( -20.18823718843633586, -278.2722409054376271, -197.2957160965913204 ) ) ;
#92115=CARTESIAN_POINT ( 'NONE',  ( 38.04568002670000482, -273.8819406966314318, -258.4678354807006144 ) ) ;
#92116=CARTESIAN_POINT ( 'NONE',  ( -24.31958225480821056, -276.2302156437014560, -342.3453661107727726 ) ) ;
#92117=CARTESIAN_POINT ( 'NONE',  ( 34.45527216119190683, -295.2899890095026194, -287.0270891889493896 ) ) ;
#92118=CARTESIAN_POINT ( 'NONE',  ( 22.64218013656804374, -279.8299477325448947, -222.5550216351258257 ) ) ;
#92119=CARTESIAN_POINT ( 'NONE',  ( -58.46468524604843253, -296.2733044206775048, -340.4840667745914402 ) ) ;
#92120=CARTESIAN_POINT ( 'NONE',  ( -97.87394220482170226, -297.2387306832472973, -317.1494278878799946 ) ) ;
#92121=CARTESIAN_POINT ( 'NONE',  ( -69.25561991581021459, -297.4534641100697741, -204.7067066431669673 ) ) ;
#92122=CARTESIAN_POINT ( 'NONE',  ( -37.58122463873551311, -294.0493461534879884, -195.3487118981795447 ) ) ;
#92123=CARTESIAN_POINT ( 'NONE',  ( -64.54917640582389993, -285.8733124002492332, -198.3139491388778026 ) ) ;
#92124=CARTESIAN_POINT ( 'NONE',  ( 25.91257838495116772, -273.1344271491331028, -228.6573803810417473 ) ) ;
#92125=CARTESIAN_POINT ( 'NONE',  ( 10.22627933519428112, -288.2501738771244959, -330.9788227866316674 ) ) ;
#92126=CARTESIAN_POINT ( 'NONE',  ( -80.01537981972640523, -281.4513914074202034, -209.1173112602517676 ) ) ;
#92127=CARTESIAN_POINT ( 'NONE',  ( -104.8096622764974342, -283.9935699379740299, -241.7442901645396205 ) ) ;
#92128=CARTESIAN_POINT ( 'NONE',  ( -81.69104272750401208, -287.6558560696544191, -330.8436481618447260 ) ) ;
#92129=CARTESIAN_POINT ( 'NONE',  ( 173.4479467868932829, 229.7134184023448142, -192.0138545908111496 ) ) ;
#92130=CARTESIAN_POINT ( 'NONE',  ( -6.985220253899331766, -285.9692186405659982, -203.8908324833523125 ) ) ;
#92132=CARTESIAN_POINT ( 'NONE',  ( -24.56091773604495998, -283.8342508652153242, -346.1083444665698039 ) ) ;
#92133=CARTESIAN_POINT ( 'NONE',  ( -61.60281816866072546, -290.8033570143372799, -197.4750708816478380 ) ) ;
#92134=CARTESIAN_POINT ( 'NONE',  ( -77.09275720576751212, -281.1293841970339145, -205.2900726959945814 ) ) ;
#92135=CARTESIAN_POINT ( 'NONE',  ( -90.72613789452995547, -280.6297838383227941, -215.4839605343739777 ) ) ;
#92136=CARTESIAN_POINT ( 'NONE',  ( 28.15013031995771087, -281.8238091456313441, -302.7220703729472007 ) ) ;
#92137=CARTESIAN_POINT ( 'NONE',  ( 29.63624354911688386, -277.1064677571801553, -236.6127001463279953 ) ) ;
#92138=CARTESIAN_POINT ( 'NONE',  ( -19.28728046576089383, -294.8261969203741728, -345.2694466029412297 ) ) ;
#92139=CARTESIAN_POINT ( 'NONE',  ( -103.8642042717651606, -289.0233785415663306, -236.3852448360190408 ) ) ;
#92140=CARTESIAN_POINT ( 'NONE',  ( -110.6832066223082194, -295.4941334381200591, -268.7122824466516136 ) ) ;
#92143=CARTESIAN_POINT ( 'NONE',  ( 8.703496828763627846, -284.3360506428081749, -328.9175981098180159 ) ) ;
#92144=CARTESIAN_POINT ( 'NONE',  ( -108.7989415408142264, -296.4178817797650254, -255.2693763011288297 ) ) ;
#92145=CARTESIAN_POINT ( 'NONE',  ( -4.748052243191166255, -293.5511440313488265, -200.9410443095753749 ) ) ;
#92146=CARTESIAN_POINT ( 'NONE',  ( -76.17425371797476430, -284.2371860237928445, -332.3558276395201574 ) ) ;
#92147=CARTESIAN_POINT ( 'NONE',  ( -29.84988571813216751, -273.2035521339015531, -193.9628658454433889 ) ) ;
#92148=CARTESIAN_POINT ( 'NONE',  ( -111.8212305396424142, -290.9631960646470361, -289.5478345414990713 ) ) ;
#92149=CARTESIAN_POINT ( 'NONE',  ( -49.12880950617137898, -284.0432150133303821, -195.4659481531978145 ) ) ;
#92150=CARTESIAN_POINT ( 'NONE',  ( -113.3385027575013311, -290.7321011129461681, -282.6179642998316126 ) ) ;
#92151=CARTESIAN_POINT ( 'NONE',  ( 14.10128641238149427, -288.6382868691399040, -322.1849216111931469 ) ) ;
#92154=CARTESIAN_POINT ( 'NONE',  ( 198.9222472290481107, 285.7997244369286705, -96.29823329932079901 ) ) ;
#92155=CARTESIAN_POINT ( 'NONE',  ( -30.25979458878175166, -284.4842132587976380, -346.3384459577605980 ) ) ;
#92156=CARTESIAN_POINT ( 'NONE',  ( 35.77081079830085031, -285.2666405000204577, -287.0812184334320705 ) ) ;
#92158=CARTESIAN_POINT ( 'NONE',  ( 21.24870238136351830, -281.0888294652893933, -314.4430737902855526 ) ) ;
#92159=CARTESIAN_POINT ( 'NONE',  ( 36.86410477721120316, -275.4760006315963778, -290.8856773332105377 ) ) ;
#92160=CARTESIAN_POINT ( 'NONE',  ( -104.7722036336553657, -280.1225945607095014, -302.9332956353616737 ) ) ;
#92161=CARTESIAN_POINT ( 'NONE',  ( 175.5294223676853562, 240.7679223315280979, -178.2279574903016623 ) ) ;
#92162=CARTESIAN_POINT ( 'NONE',  ( 38.08327240192149787, -280.2821001480572818, -282.6771018170967977 ) ) ;
#92163=CARTESIAN_POINT ( 'NONE',  ( -73.14119015358589593, -283.5952883239441462, -204.8466343622566228 ) ) ;
#92164=CARTESIAN_POINT ( 'NONE',  ( -94.80036233197064632, -297.6315636111481808, -320.0851177538386878 ) ) ;
#92165=CARTESIAN_POINT ( 'NONE',  ( 35.26881681877143393, -294.1572010639757764, -278.9115201708078757 ) ) ;
#92167=CARTESIAN_POINT ( 'NONE',  ( -107.8638171348330701, -289.5093358452252801, -249.6313410613936412 ) ) ;
#92168=CARTESIAN_POINT ( 'NONE',  ( -18.58288025350287498, -274.9389108772076042, -195.7312371196776724 ) ) ;
#92169=CARTESIAN_POINT ( 'NONE',  ( -92.91378333311681104, -273.2256387032089719, -223.0053292369560438 ) ) ;
#92171=CARTESIAN_POINT ( 'NONE',  ( -97.56176595634224213, -272.1102037436245382, -222.8738967228917716 ) ) ;
#92176=CARTESIAN_POINT ( 'NONE',  ( 5.784984827709251043, -283.5315821599924675, -329.6427771822853288 ) ) ;
#92177=CARTESIAN_POINT ( 'NONE',  ( -59.03458198338113050, -281.5353505352627508, -197.5367203637727584 ) ) ;
#92179=CARTESIAN_POINT ( 'NONE',  ( -51.07373165187753017, -282.2905828170895575, -342.3492210155351358 ) ) ;
#92180=CARTESIAN_POINT ( 'NONE',  ( 12.11133522320177036, -282.6091956308266049, -214.9963026891963693 ) ) ;
#92181=CARTESIAN_POINT ( 'NONE',  ( 23.63682128274491134, -273.4617341466191647, -228.9581937063117607 ) ) ;
#92184=CARTESIAN_POINT ( 'NONE',  ( -97.79552033249345300, -278.7195952539516952, -317.7899535576747780 ) ) ;
#92188=CARTESIAN_POINT ( 'NONE',  ( -68.48319767168499084, -285.4391456624471743, -338.9945624313600092 ) ) ;
#92189=CARTESIAN_POINT ( 'NONE',  ( -2.353237483384341022, -291.7248160040581979, -206.0941923850689363 ) ) ;
#92190=CARTESIAN_POINT ( 'NONE',  ( 37.04370229184142005, -287.1451181073712178, -289.8579047366315535 ) ) ;
#92191=CARTESIAN_POINT ( 'NONE',  ( -69.19095982766481256, -283.8671932675695189, -203.5369706117102169 ) ) ;
#92192=CARTESIAN_POINT ( 'NONE',  ( -102.7539228424638367, -283.5815338090217779, -236.6473813897290768 ) ) ;
#92193=CARTESIAN_POINT ( 'NONE',  ( 1.829139564833170528, -286.7601202057824139, -333.1593610351702637 ) ) ;
#92194=CARTESIAN_POINT ( 'NONE',  ( -107.7686164525559889, -285.4847289093170843, -291.0742913940970880 ) ) ;
#92195=CARTESIAN_POINT ( 'NONE',  ( 35.94575831833729040, -273.7573775859350462, -286.3568093329479325 ) ) ;
#92196=CARTESIAN_POINT ( 'NONE',  ( 38.18507422594242939, -285.8243005830075276, -260.2543494226483176 ) ) ;
#92197=CARTESIAN_POINT ( 'NONE',  ( -100.6423988056475878, -299.0935691335796491, -230.1364713737373791 ) ) ;
#92198=CARTESIAN_POINT ( 'NONE',  ( -92.55533242118022486, -283.2641184400021643, -219.2801281553609556 ) ) ;
#92199=CARTESIAN_POINT ( 'NONE',  ( -14.24600351129383569, -281.3002647426362728, -200.8093280125607123 ) ) ;
#92200=CARTESIAN_POINT ( 'NONE',  ( 34.92145991046990616, -289.2844816226241278, -249.4868153894530280 ) ) ;
#92203=CARTESIAN_POINT ( 'NONE',  ( -101.8728308340789681, -297.9492272323626594, -309.6682085169498464 ) ) ;
#92204=CARTESIAN_POINT ( 'NONE',  ( -43.90130609867937039, -277.9692035606338436, -195.5969103175798693 ) ) ;
#92205=CARTESIAN_POINT ( 'NONE',  ( -102.1705312572491664, -289.2064142907390192, -311.7068565704846037 ) ) ;
#92206=CARTESIAN_POINT ( 'NONE',  ( 4.250634731313062353, -292.8808198747910865, -331.3243699842163323 ) ) ;
#92207=CARTESIAN_POINT ( 'NONE',  ( -38.34386269574050488, -278.7241583040062096, -196.8623143927832473 ) ) ;
#92208=CARTESIAN_POINT ( 'NONE',  ( -58.23003210534655949, -295.9188985158894525, -199.1252908642997852 ) ) ;
#92209=CARTESIAN_POINT ( 'NONE',  ( 13.23045453135390304, -294.0926145982928119, -217.0347581752882604 ) ) ;
#92210=CARTESIAN_POINT ( 'NONE',  ( -4.829096099716510437, -288.9805209788416391, -202.7746430608542312 ) ) ;
#92211=CARTESIAN_POINT ( 'NONE',  ( -110.1457271592157241, -295.3237972234453537, -247.3326282225894488 ) ) ;
#92212=CARTESIAN_POINT ( 'NONE',  ( -78.60502091279583681, -291.2178118523368084, -331.6090555798036235 ) ) ;
#92213=CARTESIAN_POINT ( 'NONE',  ( 32.40330115951777401, -291.4025775502460078, -240.2013963849918241 ) ) ;
#92214=CARTESIAN_POINT ( 'NONE',  ( -107.5084575424834128, -291.6837493782022648, -292.7106225379789066 ) ) ;
#92215=ADVANCED_FACE ( 'NONE', ( #76567 ), #23607, .F. ) ;
#92217=CARTESIAN_POINT ( 'NONE',  ( -95.24845408909473576, -291.9831262664929454, -225.6463600921897807 ) ) ;
#92219=CARTESIAN_POINT ( 'NONE',  ( -113.9720259457677258, -291.7821268469442657, -268.3803722770622926 ) ) ;
#92220=CARTESIAN_POINT ( 'NONE',  ( 0.5687818237891290041, -278.5745202268709022, -205.1771869677942277 ) ) ;
#92221=CARTESIAN_POINT ( 'NONE',  ( 29.85574526842174947, -293.1676665568263047, -241.7098139173920401 ) ) ;
#92222=CARTESIAN_POINT ( 'NONE',  ( -39.58725916897031283, -280.0247176494351038, -193.3808179989841847 ) ) ;
#92223=CARTESIAN_POINT ( 'NONE',  ( -111.8555693876049872, -283.9763558657629119, -289.7376626467539040 ) ) ;
#92224=CARTESIAN_POINT ( 'NONE',  ( 23.43617371858514886, -286.1473971568800039, -314.0197766768680481 ) ) ;
#92225=CARTESIAN_POINT ( 'NONE',  ( 33.92696323495075461, -279.4214710237247346, -249.5850956529434370 ) ) ;
#92226=CARTESIAN_POINT ( 'NONE',  ( -33.79572641913322428, -284.0966204441852483, -195.4449867343163021 ) ) ;
#92227=CARTESIAN_POINT ( 'NONE',  ( 28.69632656350021804, -279.5303523302633266, -232.1291054537108778 ) ) ;
#92228=CARTESIAN_POINT ( 'NONE',  ( 21.86035610847062571, -285.8148781798079767, -221.6106405654452089 ) ) ;
#92230=CARTESIAN_POINT ( 'NONE',  ( 15.43350097081438754, -294.4132564806113237, -218.7009453128011671 ) ) ;
#92231=CARTESIAN_POINT ( 'NONE',  ( 38.72885893514061451, -276.8798855086320145, -262.6218382784726373 ) ) ;
#92232=CARTESIAN_POINT ( 'NONE',  ( -24.33000313824093297, -276.5482964787728406, -342.2650934989455891 ) ) ;
#92233=CARTESIAN_POINT ( 'NONE',  ( -112.6404178736079587, -290.9208841501561551, -254.2022223462749366 ) ) ;
#92234=CARTESIAN_POINT ( 'NONE',  ( -27.58277256195642835, -281.0090946815363964, -345.3406282654490269 ) ) ;
#92236=CARTESIAN_POINT ( 'NONE',  ( -107.9756624265907163, -289.8656723942427789, -251.0155288570420851 ) ) ;
#92237=CARTESIAN_POINT ( 'NONE',  ( -92.24326195022581487, -293.8367803861256675, -321.4762157344185880 ) ) ;
#92239=CARTESIAN_POINT ( 'NONE',  ( -14.82148196441097454, -291.8596224417491953, -200.8569582839153043 ) ) ;
#92242=CARTESIAN_POINT ( 'NONE',  ( 7.450504543161054372, -272.1952119285918457, -214.2458315076590907 ) ) ;
#92243=CARTESIAN_POINT ( 'NONE',  ( -105.0404320084053182, -296.0812981215323703, -234.0585842990633694 ) ) ;
#92244=CARTESIAN_POINT ( 'NONE',  ( 36.65396876758700273, -279.8993900819789360, -286.6981247717925498 ) ) ;
#92245=CARTESIAN_POINT ( 'NONE',  ( -113.0023115558056332, -286.0145593653165861, -258.6635762973609189 ) ) ;
#92246=CARTESIAN_POINT ( 'NONE',  ( -35.93133902273247315, -285.9036501387922158, -197.3747433220484311 ) ) ;
#92247=CARTESIAN_POINT ( 'NONE',  ( 1.250861165908237371, -278.0471246036970001, -333.2010361074588332 ) ) ;
#92248=CARTESIAN_POINT ( 'NONE',  ( -105.4474449543378825, -294.1683133094104505, -301.0400487017277555 ) ) ;
#92249=CARTESIAN_POINT ( 'NONE',  ( -108.8200541069438003, -298.5630527555596814, -251.1075652290759592 ) ) ;
#92250=CARTESIAN_POINT ( 'NONE',  ( -100.9344959331764073, -276.8460881183456195, -307.1113789955583115 ) ) ;
#92253=CARTESIAN_POINT ( 'NONE',  ( -112.8671136782256070, -296.4059681149219045, -255.4052258804949815 ) ) ;
#92254=CARTESIAN_POINT ( 'NONE',  ( 29.53190838839401167, -289.9066480218052675, -303.0602720826641985 ) ) ;
#92256=CARTESIAN_POINT ( 'NONE',  ( 28.32295606611701189, -288.6381113537674423, -302.4865844340063745 ) ) ;
#92258=CARTESIAN_POINT ( 'NONE',  ( -71.12022602912675495, -278.6759169596537049, -201.4275891154477449 ) ) ;
#92259=CARTESIAN_POINT ( 'NONE',  ( -111.5259488317175851, -297.4597361964793549, -249.9155729426356629 ) ) ;
#92260=CARTESIAN_POINT ( 'NONE',  ( -110.7911859833681234, -288.9287032777452850, -251.7218752484802735 ) ) ;
#92261=CARTESIAN_POINT ( 'NONE',  ( -114.2124237528593511, -296.8231197402293446, -275.3422355777246935 ) ) ;
#92262=CARTESIAN_POINT ( 'NONE',  ( 33.46760488580594028, -294.1207624177496882, -288.1973118116284240 ) ) ;
#92266=CARTESIAN_POINT ( 'NONE',  ( 32.24064525209211496, -289.4759654089318701, -301.6821167265741224 ) ) ;
#92267=CARTESIAN_POINT ( 'NONE',  ( -99.90806341382572953, -281.6948066931272479, -220.5068182859052968 ) ) ;
#92269=CARTESIAN_POINT ( 'NONE',  ( 26.20107647552291041, -280.3277403440131934, -226.9596683785739799 ) ) ;
#92270=CARTESIAN_POINT ( 'NONE',  ( -92.06517812412242563, -285.8362080835908046, -321.4039370950949888 ) ) ;
#92272=CARTESIAN_POINT ( 'NONE',  ( 25.88012464252941669, -285.5564764560488697, -227.4237860734758954 ) ) ;
#92273=CARTESIAN_POINT ( 'NONE',  ( -111.7467798112649433, -288.5855052615702334, -273.9545584431152179 ) ) ;
#92274=CARTESIAN_POINT ( 'NONE',  ( 38.39547106792315390, -277.3865629595952669, -268.3150541804079694 ) ) ;
#92276=CARTESIAN_POINT ( 'NONE',  ( -108.4862654471839960, -278.3356859625646393, -286.7704393067185720 ) ) ;
#92277=CARTESIAN_POINT ( 'NONE',  ( 35.13497451868102672, -280.7700919818917100, -260.4437811557052669 ) ) ;
#92278=CARTESIAN_POINT ( 'NONE',  ( 38.43252789911300482, -276.7844557826115306, -282.5167594656351753 ) ) ;
#92279=CARTESIAN_POINT ( 'NONE',  ( -59.17421544043035198, -278.5706110470615045, -196.9353051318821315 ) ) ;
#92280=CARTESIAN_POINT ( 'NONE',  ( 101.3885564533947132, 116.0994877786729944, -280.6488961443201902 ) ) ;
#92281=CARTESIAN_POINT ( 'NONE',  ( -49.69323055338989548, -274.8396986135285829, -194.5429730840638172 ) ) ;
#92282=CARTESIAN_POINT ( 'NONE',  ( -108.5268680866647486, -274.4252176589839110, -242.7314046901510949 ) ) ;
#92283=CARTESIAN_POINT ( 'NONE',  ( -106.6662871844225293, -287.4805209788416391, -237.0123917617630980 ) ) ;
#92284=CARTESIAN_POINT ( 'NONE',  ( 129.9467878515196162, -299.5541904835127980, -200.7046326357662167 ) ) ;
#92285=CARTESIAN_POINT ( 'NONE',  ( 31.25901186464348669, -288.2866270422087496, -244.3689389846792892 ) ) ;
#92286=CARTESIAN_POINT ( 'NONE',  ( 22.18389846867367865, -288.6715833538992797, -223.1103425658456558 ) ) ;
#92287=CARTESIAN_POINT ( 'NONE',  ( 28.31568157913729777, -287.3354945827409210, -302.5014492686228778 ) ) ;
#92288=CARTESIAN_POINT ( 'NONE',  ( -110.8653598411162307, -284.3467323289016804, -247.5147273865749469 ) ) ;
#92289=CARTESIAN_POINT ( 'NONE',  ( -70.07699919036306824, -278.0133875953563347, -204.2045452565980383 ) ) ;
#92290=CARTESIAN_POINT ( 'NONE',  ( -49.64925598126998807, -287.7541078901966216, -197.1008938015943102 ) ) ;
#92291=CARTESIAN_POINT ( 'NONE',  ( 11.78226379117393208, -279.2292019679542250, -215.4289423501730596 ) ) ;
#92292=CARTESIAN_POINT ( 'NONE',  ( -59.32667500354519063, -278.6579949677140462, -340.4888896342499152 ) ) ;
#92293=CARTESIAN_POINT ( 'NONE',  ( -32.41014727835776199, -277.4807887021507895, -343.3060384995462755 ) ) ;
#92294=CARTESIAN_POINT ( 'NONE',  ( -40.33866810305801920, -287.8839397658408075, -346.9184127381960252 ) ) ;
#92295=CARTESIAN_POINT ( 'NONE',  ( 19.67058461752129261, -283.0566368584561019, -321.9536152058485641 ) ) ;
#92296=CARTESIAN_POINT ( 'NONE',  ( -112.1578352728291463, -284.8191745609818781, -288.3632571558972586 ) ) ;
#92297=CARTESIAN_POINT ( 'NONE',  ( 24.13158749145670257, -282.2645867068694088, -309.8245316795982376 ) ) ;
#92300=CARTESIAN_POINT ( 'NONE',  ( 121.3395553409046528, -296.8152984961567427, -195.3611179825600175 ) ) ;
#92301=CARTESIAN_POINT ( 'NONE',  ( -110.8028588639680123, -292.6489333521008689, -251.7679302346301711 ) ) ;
#92302=CARTESIAN_POINT ( 'NONE',  ( -40.59458186991012241, -290.6969084256586484, -193.9103524594466990 ) ) ;
#92303=CARTESIAN_POINT ( 'NONE',  ( -72.00855973548746647, -272.6409959338194540, -205.7940179997810048 ) ) ;
#92304=CARTESIAN_POINT ( 'NONE',  ( 37.35900325008093148, -293.1299764320229997, -288.6677030066111342 ) ) ;
#92306=CARTESIAN_POINT ( 'NONE',  ( -40.00235977253007036, -287.5659332485013238, -344.0564582181897322 ) ) ;
#92307=CARTESIAN_POINT ( 'NONE',  ( 32.76805845636194192, -291.4793028913970829, -246.4823313087376846 ) ) ;
#92309=CARTESIAN_POINT ( 'NONE',  ( -39.95682695602013013, -290.2906886463000546, -343.7614352514647180 ) ) ;
#92310=DIRECTION ( 'NONE',  ( 0.000000000000000000, 0.000000000000000000, 1.000000000000000000 ) ) ;
#92311=CARTESIAN_POINT ( 'NONE',  ( -92.11430713159376182, -291.8342549182078756, -321.6703205373823948 ) ) ;
#92312=CARTESIAN_POINT ( 'NONE',  ( -94.25569371910715688, -289.2314237010997999, -221.2412922283180308 ) ) ;
#92314=CARTESIAN_POINT ( 'NONE',  ( -79.00362692893637018, -293.4909826529812449, -207.9352936989693603 ) ) ;
#92315=CARTESIAN_POINT ( 'NONE',  ( 13.29360894974098173, -287.7224703606501635, -217.3811099711532790 ) ) ;
#92316=CARTESIAN_POINT ( 'NONE',  ( 26.48189180133820031, -295.0190670001029503, -230.5566810147311685 ) ) ;
#92319=CARTESIAN_POINT ( 'NONE',  ( -5.825641502940878347, -276.4443388915217383, -201.9129999996004017 ) ) ;
#92320=CARTESIAN_POINT ( 'NONE',  ( -113.9589469772315908, -295.8306235535918631, -263.8738918065893131 ) ) ;
#92321=CARTESIAN_POINT ( 'NONE',  ( 1.158457435358022369, -272.8137145038447784, -207.1494744294204509 ) ) ;
#92322=CARTESIAN_POINT ( 'NONE',  ( -107.7999268318789632, -276.9468911568533827, -246.1831459873743313 ) ) ;
#92323=CARTESIAN_POINT ( 'NONE',  ( -87.61640209655796241, -274.5366816873591915, -216.8164309816662580 ) ) ;
#92324=CARTESIAN_POINT ( 'NONE',  ( -90.82307977799618470, -297.2544374603523352, -320.9826472191942912 ) ) ;
#92326=CARTESIAN_POINT ( 'NONE',  ( -104.9152558011691241, -297.7302119871392279, -242.3180029591451330 ) ) ;
#92328=CARTESIAN_POINT ( 'NONE',  ( 15.17142995382244486, -284.8091770220731860, -216.3168956254932027 ) ) ;
#92329=CARTESIAN_POINT ( 'NONE',  ( -68.04752391275964385, -297.6374348207216372, -204.1194202711456569 ) ) ;
#92330=CARTESIAN_POINT ( 'NONE',  ( -60.50992131055743073, -285.7598909318557503, -196.8737128612835079 ) ) ;
#92331=CARTESIAN_POINT ( 'NONE',  ( -37.50580642586700009, -288.7208385459273927, -347.3528673581230919 ) ) ;
#92332=CARTESIAN_POINT ( 'NONE',  ( -96.10852583545484151, -297.8859912694574632, -317.5500273586097819 ) ) ;
#92333=CARTESIAN_POINT ( 'NONE',  ( 22.78468102161714981, -292.1613886565898497, -314.9127365726932908 ) ) ;
#92334=CARTESIAN_POINT ( 'NONE',  ( 15.05870482382987596, -279.9659114116985279, -214.0891177953703561 ) ) ;
#92335=CARTESIAN_POINT ( 'NONE',  ( -85.28047601435908120, -288.9094976428776818, -210.1954327657594206 ) ) ;
#92337=CARTESIAN_POINT ( 'NONE',  ( -42.70818369039324125, -287.9161411897082417, -343.6126213517956671 ) ) ;
#92339=CARTESIAN_POINT ( 'NONE',  ( 11.39612404223932351, -286.3767784449806868, -327.4352506789019230 ) ) ;
#92340=CARTESIAN_POINT ( 'NONE',  ( -68.40260495460989887, -299.2373038247618524, -203.4020963817534096 ) ) ;
#92341=CARTESIAN_POINT ( 'NONE',  ( -48.05426540342109121, -281.3438325209871778, -194.6515723423923134 ) ) ;
#92342=CARTESIAN_POINT ( 'NONE',  ( -111.7611038063295013, -294.7245969887872548, -258.4406608521890121 ) ) ;
#92343=CARTESIAN_POINT ( 'NONE',  ( 19.35203898731771233, -282.2030330379161569, -316.3679929442639605 ) ) ;
#92344=CARTESIAN_POINT ( 'NONE',  ( -110.8137658269120607, -297.0103271155928155, -247.1440507521128609 ) ) ;
#92345=CARTESIAN_POINT ( 'NONE',  ( -105.9722901025433828, -274.3310865244872048, -243.6645393570520923 ) ) ;
#92346=CARTESIAN_POINT ( 'NONE',  ( 15.78786429297873006, -282.8041539373235764, -217.3520389658156660 ) ) ;
#92347=CARTESIAN_POINT ( 'NONE',  ( -67.17074346553154385, -272.5719656088507463, -203.3813005540561960 ) ) ;
#92350=CARTESIAN_POINT ( 'NONE',  ( -68.44730547988727665, -285.4427669884234433, -338.2160229043689696 ) ) ;
#92352=CARTESIAN_POINT ( 'NONE',  ( -69.85430415644619018, -289.1237833571632905, -202.7746430608542312 ) ) ;
#92353=CARTESIAN_POINT ( 'NONE',  ( 19.75035846940255979, -275.4490506322395049, -321.8070212831317463 ) ) ;
#92354=CARTESIAN_POINT ( 'NONE',  ( 8.850481388264096694, -292.5392735307085559, -213.7687220435549023 ) ) ;
#92355=CARTESIAN_POINT ( 'NONE',  ( 19.03717703127611927, -283.7402298262488216, -317.8373246556525373 ) ) ;
#92356=CARTESIAN_POINT ( 'NONE',  ( 35.15560644665041679, -276.9721454594476313, -256.5560118213106193 ) ) ;
#92357=CARTESIAN_POINT ( 'NONE',  ( -113.3160529357301556, -285.8746459840568264, -278.5161169109562707 ) ) ;
#92358=CARTESIAN_POINT ( 'NONE',  ( -5.876569458893204256, -281.4240098572850570, -336.6853941419780085 ) ) ;
#92359=CARTESIAN_POINT ( 'NONE',  ( -105.1897154986274074, -280.9740806400527049, -238.2757403489738977 ) ) ;
#92360=CARTESIAN_POINT ( 'NONE',  ( 33.71272902355963907, -275.3399628929311689, -240.5541036817906786 ) ) ;
#92361=CARTESIAN_POINT ( 'NONE',  ( 38.21915848302209184, -275.2001603839090649, -255.5436738548442293 ) ) ;
#92362=CARTESIAN_POINT ( 'NONE',  ( -34.21674308949055643, -296.9327062603370564, -344.7355009611281957 ) ) ;
#92365=CARTESIAN_POINT ( 'NONE',  ( -66.47178800654958764, -293.5691398486422941, -340.3160939247162560 ) ) ;
#92366=CARTESIAN_POINT ( 'NONE',  ( 0.8982964622461634407, -276.0349798733692523, -332.6756102250192839 ) ) ;
#92367=AXIS2_PLACEMENT_3D ( 'NONE', #66873, #89088, #45529 ) ;
#92368=CARTESIAN_POINT ( 'NONE',  ( 23.48809492524796738, -295.6915857997874468, -316.4311059189952857 ) ) ;
#92369=CARTESIAN_POINT ( 'NONE',  ( -4.657948827176248585, -295.8362059009780296, -339.6559675273774133 ) ) ;
#92371=CARTESIAN_POINT ( 'NONE',  ( -75.94668771473020286, -293.5358917652927175, -206.1937969760872136 ) ) ;
#92373=CARTESIAN_POINT ( 'NONE',  ( -99.17774930438719139, -275.9800244522102162, -312.5076652827130488 ) ) ;
#92374=CARTESIAN_POINT ( 'NONE',  ( -109.6949650857145286, -280.6987555229260352, -252.8591394829081764 ) ) ;
#92375=CARTESIAN_POINT ( 'NONE',  ( -93.28878772601973424, -293.9446465654510803, -319.4654720558318672 ) ) ;
#92376=CARTESIAN_POINT ( 'NONE',  ( 31.28380535012820118, -283.8317752433003989, -302.5915855325646930 ) ) ;
#92377=CARTESIAN_POINT ( 'NONE',  ( -41.32603987864296613, -284.9211706674892639, -197.1478076631026397 ) ) ;
#92378=CARTESIAN_POINT ( 'NONE',  ( -29.18771587708346615, -125.5003645754393915, -363.4224408895635747 ) ) ;
#92380=CARTESIAN_POINT ( 'NONE',  ( -109.6325590332666309, -284.3547228059580902, -260.0597003358899997 ) ) ;
#92382=CARTESIAN_POINT ( 'NONE',  ( 32.88435712544961120, -282.2371944979362297, -239.5423997818317048 ) ) ;
#92383=CARTESIAN_POINT ( 'NONE',  ( -113.9290005361301752, -283.3878749898391334, -267.1158424668637394 ) ) ;
#92384=CARTESIAN_POINT ( 'NONE',  ( -111.8604135686670560, -279.7253183986641147, -251.8739877468008217 ) ) ;
#92385=CARTESIAN_POINT ( 'NONE',  ( -92.81651322988420816, -279.3496176672071556, -322.8320783532010410 ) ) ;
#92386=CARTESIAN_POINT ( 'NONE',  ( -82.18614792566211236, -280.1093904727838435, -207.8928197183208795 ) ) ;
#92387=CARTESIAN_POINT ( 'NONE',  ( -67.74223827176246004, -274.9809262143061233, -333.4151289067050357 ) ) ;
#92388=CARTESIAN_POINT ( 'NONE',  ( -98.94016388745465918, -248.7537405824094208, -334.3288800165568659 ) ) ;
#92390=CARTESIAN_POINT ( 'NONE',  ( -16.14516622885952657, -276.3268667587246910, -198.5384683514388087 ) ) ;
#92391=CARTESIAN_POINT ( 'NONE',  ( -64.16662707700760393, -182.5074878589848026, -362.2231175211663299 ) ) ;
#92392=CARTESIAN_POINT ( 'NONE',  ( -93.42800663272525696, -277.2600484248416137, -221.0854839873903757 ) ) ;
#92393=CARTESIAN_POINT ( 'NONE',  ( -1.304463679438762069, -294.2836156537364900, -203.4634976634465318 ) ) ;
#92394=CARTESIAN_POINT ( 'NONE',  ( 18.04424157008249807, -293.5794663659752928, -318.0906837000248402 ) ) ;
#92395=CARTESIAN_POINT ( 'NONE',  ( -80.51127564382603907, -289.1276099087729108, -334.1115455632428279 ) ) ;
#92397=CARTESIAN_POINT ( 'NONE',  ( -11.27540808798117844, -293.2939136892524061, -342.2445051051164455 ) ) ;
#92398=CARTESIAN_POINT ( 'NONE',  ( -84.13960492805603053, -283.7965362980150985, -213.2298892644596435 ) ) ;
#92399=CARTESIAN_POINT ( 'NONE',  ( -70.79826222694117632, -293.4663746965425730, -204.0925437123178483 ) ) ;
#92400=CARTESIAN_POINT ( 'NONE',  ( -94.51618866481463499, -286.5161646675685461, -224.1641012833078719 ) ) ;
#92402=CARTESIAN_POINT ( 'NONE',  ( -66.93584214508034336, -292.6148942695525079, -199.5302845020301561 ) ) ;
#92403=CARTESIAN_POINT ( 'NONE',  ( -56.32885733811063034, -283.7958517097265485, -340.9123497404513046 ) ) ;
#92404=CARTESIAN_POINT ( 'NONE',  ( -16.62907155743504006, -293.5853953982571056, -344.1656097387794375 ) ) ;
#92405=CARTESIAN_POINT ( 'NONE',  ( 22.28632056984372056, -289.0067130362657508, -318.8447835755719666 ) ) ;
#92406=CARTESIAN_POINT ( 'NONE',  ( -51.66769595194030984, -289.7230598291117758, -345.9540590995590605 ) ) ;
#92407=CARTESIAN_POINT ( 'NONE',  ( 34.56702236190806588, -287.5491843030301879, -257.5008271373959587 ) ) ;
#92410=CARTESIAN_POINT ( 'NONE',  ( -89.83885599784697717, -297.6436107370255399, -325.0625676247297520 ) ) ;
#92411=CARTESIAN_POINT ( 'NONE',  ( -54.46838210687174353, -296.5213727501273979, -195.7958778514147582 ) ) ;
#92412=CARTESIAN_POINT ( 'NONE',  ( 2.843076177543889305, -279.6644179167183211, -209.0745134814166590 ) ) ;
#92413=CARTESIAN_POINT ( 'NONE',  ( -55.31315761928669872, -273.3345801644555877, -195.5510008947174470 ) ) ;
#92414=CARTESIAN_POINT ( 'NONE',  ( -58.62682165520693189, -293.8123267978988338, -340.9135903176421039 ) ) ;
#92415=CARTESIAN_POINT ( 'NONE',  ( 33.82829857066034407, -277.0451818656903242, -249.8605770083961772 ) ) ;
#92416=CARTESIAN_POINT ( 'NONE',  ( -70.01359868815212906, -271.7566574197194313, -203.7021911362464834 ) ) ;
#92417=CARTESIAN_POINT ( 'NONE',  ( -12.86141856604536571, -295.9319840631955572, -339.6089355899658813 ) ) ;
#92418=CARTESIAN_POINT ( 'NONE',  ( -35.62966877391741605, -296.1098791767777811, -343.6627862385698791 ) ) ;
#92420=CARTESIAN_POINT ( 'NONE',  ( -6.106797634887838555, -296.2486052104973737, -339.8652278160894866 ) ) ;
#92421=CARTESIAN_POINT ( 'NONE',  ( -94.21152794698913624, -293.8718696533530306, -319.5124263356717620 ) ) ;
#92422=CARTESIAN_POINT ( 'NONE',  ( -47.01615458380901202, -292.5774353946418387, -197.9021806525712179 ) ) ;
#92423=CARTESIAN_POINT ( 'NONE',  ( -49.70335915969832996, -274.7013014873882071, -194.4697808734456430 ) ) ;
#92424=CARTESIAN_POINT ( 'NONE',  ( -110.2816767919995868, -289.2594485418899239, -260.2301535650274218 ) ) ;
#92425=CARTESIAN_POINT ( 'NONE',  ( -40.89449690936561410, -276.0077436718352715, -195.3942487085843993 ) ) ;
#92426=CARTESIAN_POINT ( 'NONE',  ( -114.1200850071242030, -273.1161426097481808, -264.6370713041806653 ) ) ;
#92427=CARTESIAN_POINT ( 'NONE',  ( -68.06028761040789732, -297.9706619686879208, -204.1020277631467081 ) ) ;
#92428=CARTESIAN_POINT ( 'NONE',  ( -83.57803754824804798, -281.4018631775118706, -210.7920609206440474 ) ) ;
#92429=CARTESIAN_POINT ( 'NONE',  ( -2.599025925956609751, -279.1866888084022094, -202.1831143562232285 ) ) ;
#92430=CARTESIAN_POINT ( 'NONE',  ( -35.72198420555046283, -276.3809561960087535, -347.2552317297560194 ) ) ;
#92431=CARTESIAN_POINT ( 'NONE',  ( 0.9893635474065419766, -278.9542227553109228, -204.4438417663529890 ) ) ;
#92432=CARTESIAN_POINT ( 'NONE',  ( 14.47094055627969844, -280.3251422888931756, -324.8173269029031189 ) ) ;
#92433=CARTESIAN_POINT ( 'NONE',  ( -13.86038227978747805, -272.9376484031900532, -200.6187160415323092 ) ) ;
#92434=CARTESIAN_POINT ( 'NONE',  ( -96.50257124089317529, -279.9198143362530118, -316.4792577836873875 ) ) ;
#92437=CARTESIAN_POINT ( 'NONE',  ( -72.78770741631151964, -295.8294909808643638, -203.0903015163875409 ) ) ;
#92438=CARTESIAN_POINT ( 'NONE',  ( 20.07395324843201578, -290.8997583614815312, -221.5372004775421715 ) ) ;
#92440=CARTESIAN_POINT ( 'NONE',  ( -42.05396223094423647, -291.9942947593717690, -193.5054442435709916 ) ) ;
#92441=CARTESIAN_POINT ( 'NONE',  ( 24.57163989498581813, -278.1297590531165724, -313.0747946223415283 ) ) ;
#92442=CARTESIAN_POINT ( 'NONE',  ( -32.53817334128842731, -272.1125250108581781, -195.5022281464653986 ) ) ;
#92443=DIRECTION ( 'NONE',  ( -1.000000000000000000, -0.000000000000000000, -0.000000000000000000 ) ) ;
#92444=CARTESIAN_POINT ( 'NONE',  ( 33.25105002310052527, -283.8199065750541195, -297.3050936023727218 ) ) ;
#92446=CARTESIAN_POINT ( 'NONE',  ( -38.72469510748567956, -284.0346815335708470, -195.3612413815589832 ) ) ;
#92448=CARTESIAN_POINT ( 'NONE',  ( -53.25031351071658747, -294.0555033401352603, -342.0656486522744899 ) ) ;
#92449=CARTESIAN_POINT ( 'NONE',  ( 36.34751924726685957, -285.8083108793463794, -279.3480210927828011 ) ) ;
#92451=CARTESIAN_POINT ( 'NONE',  ( -20.42106327112575315, -292.8348034784260676, -343.4810037941167025 ) ) ;
#92452=CARTESIAN_POINT ( 'NONE',  ( -107.2828137259667898, -283.4260554701794490, -239.7176304780192595 ) ) ;
#92453=CARTESIAN_POINT ( 'NONE',  ( -90.05916104119076238, -280.8923796812117075, -218.6426686473634220 ) ) ;
#92454=CARTESIAN_POINT ( 'NONE',  ( -67.04930770811191110, -286.8763560446274710, -199.7532800959490373 ) ) ;
#92455=CARTESIAN_POINT ( 'NONE',  ( 38.26740856491498022, -279.8943142389313721, -278.4334528982410575 ) ) ;
#92456=CARTESIAN_POINT ( 'NONE',  ( 33.02926598127910296, -287.2956113131820075, -250.9465067622640504 ) ) ;
#92457=CARTESIAN_POINT ( 'NONE',  ( -101.0842191552740559, -279.4760126265431381, -307.2365895810415282 ) ) ;
#92458=CARTESIAN_POINT ( 'NONE',  ( -97.77646495367817181, -278.7825651350120779, -311.5950958110067290 ) ) ;
#92459=CARTESIAN_POINT ( 'NONE',  ( -31.04692836020613100, -288.1111822576340842, -195.2562791383247145 ) ) ;
#92461=CARTESIAN_POINT ( 'NONE',  ( 99.18810204040222800, -299.5506171838408136, -193.3647305641561047 ) ) ;
#92462=CARTESIAN_POINT ( 'NONE',  ( -111.4187789823227774, -292.4135038073661690, -279.5498714609097988 ) ) ;
#92463=CARTESIAN_POINT ( 'NONE',  ( -111.2869819898779866, -293.4805209788416391, -234.7871824221999191 ) ) ;
#92465=CARTESIAN_POINT ( 'NONE',  ( -21.71057506694973682, -272.2519085613607785, -196.8376771436088859 ) ) ;
#92466=CARTESIAN_POINT ( 'NONE',  ( -110.4536339652047303, -294.6793314764457818, -291.8800870402612304 ) ) ;
#92467=CARTESIAN_POINT ( 'NONE',  ( 94.55604251903913848, -299.2547878850892289, -197.3111030628182903 ) ) ;
#92468=CARTESIAN_POINT ( 'NONE',  ( 31.13656435624857721, -289.4347994536315127, -297.7281449038080723 ) ) ;
#92469=CARTESIAN_POINT ( 'NONE',  ( -7.612708556557906014, -282.2074094431987987, -202.5670169396713902 ) ) ;
#92470=CARTESIAN_POINT ( 'NONE',  ( -100.1855814773067976, -291.3989491297747918, -313.8266545614586676 ) ) ;
#92471=CARTESIAN_POINT ( 'NONE',  ( -109.3954133496011849, -291.5387920046486556, -296.2389033494619071 ) ) ;
#92472=CARTESIAN_POINT ( 'NONE',  ( -37.30477823177420760, -288.0527346064550898, -195.3483429767250925 ) ) ;
#92473=CARTESIAN_POINT ( 'NONE',  ( -36.75468551780674886, -280.2260185924430402, -193.3503100811241211 ) ) ;
#92474=CARTESIAN_POINT ( 'NONE',  ( -36.31893663002138339, -293.1193119070928219, -345.9270587204782146 ) ) ;
#92475=CARTESIAN_POINT ( 'NONE',  ( 29.76085774804294104, -281.8766870924667955, -308.2354617066612832 ) ) ;
#92476=CARTESIAN_POINT ( 'NONE',  ( 21.83568164135893142, -278.0319096686571925, -315.1819052347053685 ) ) ;
#92478=CARTESIAN_POINT ( 'NONE',  ( -106.6379572354042296, -298.6233781216988632, -303.7686719486574702 ) ) ;
#92479=CARTESIAN_POINT ( 'NONE',  ( 9.878578092673036437, -274.6522206064715306, -329.9616376689355661 ) ) ;
#92481=CARTESIAN_POINT ( 'NONE',  ( 18.01525293269430250, -280.3811044283108345, -222.6596693763912356 ) ) ;
#92482=CARTESIAN_POINT ( 'NONE',  ( -111.0542265122078760, -279.4946281539255892, -291.2051140777136311 ) ) ;
#92483=CARTESIAN_POINT ( 'NONE',  ( -110.3777054418884518, -273.9745742520231033, -262.1766567663059959 ) ) ;
#92484=CARTESIAN_POINT ( 'NONE',  ( -91.72781268998785720, -284.3583672805116862, -216.1857455974873119 ) ) ;
#92485=CARTESIAN_POINT ( 'NONE',  ( -99.68339717852953186, -291.7680111256601094, -310.2545613256325510 ) ) ;
#92486=CARTESIAN_POINT ( 'NONE',  ( -73.58253832576244235, -275.1799639612625583, -203.2722967066240471 ) ) ;
#92487=CARTESIAN_POINT ( 'NONE',  ( -113.3744484654679496, -273.9743643694620800, -261.8570335280117547 ) ) ;
#92489=CARTESIAN_POINT ( 'NONE',  ( 22.46461596077932299, -275.9702737849684695, -312.3072407396416565 ) ) ;
#92490=CARTESIAN_POINT ( 'NONE',  ( -111.6211050277696870, -298.4300368581620546, -279.8632869663230167 ) ) ;
#92491=CARTESIAN_POINT ( 'NONE',  ( -93.96256545681870875, -281.8717741524594658, -319.3102295882197836 ) ) ;
#92492=CARTESIAN_POINT ( 'NONE',  ( -108.3459963112656084, -290.5971806542126501, -240.6267235045343966 ) ) ;
#92493=CARTESIAN_POINT ( 'NONE',  ( 34.82610822964737451, -273.8185249060819615, -289.4308385419566889 ) ) ;
#92494=CARTESIAN_POINT ( 'NONE',  ( 36.01980672278555318, -289.4137326234675811, -291.0131357640676697 ) ) ;
#92495=CARTESIAN_POINT ( 'NONE',  ( -110.6159212601936872, -289.4258526416617201, -273.9102701976490266 ) ) ;
#92497=CARTESIAN_POINT ( 'NONE',  ( -113.0795934929261648, -289.2592741451185816, -259.8562414806100946 ) ) ;
#92498=CARTESIAN_POINT ( 'NONE',  ( -92.56970891164738191, -290.8993613513613923, -222.5913102308176690 ) ) ;
#92500=CARTESIAN_POINT ( 'NONE',  ( 7.352582380548118302, -287.7250305501481762, -207.9746668260836202 ) ) ;
#92501=CARTESIAN_POINT ( 'NONE',  ( -67.31884827615527911, -279.9811627624397374, -203.7632894113078805 ) ) ;
#92503=CARTESIAN_POINT ( 'NONE',  ( -58.77815523803668185, -294.2432934187202704, -344.0505035224324502 ) ) ;
#92504=CARTESIAN_POINT ( 'NONE',  ( -52.88888448907410123, -283.8976531718593606, -345.7255481955066330 ) ) ;
#92505=CARTESIAN_POINT ( 'NONE',  ( -64.54369072844005473, -286.0398866648573630, -198.3344827668701100 ) ) ;
#92506=CARTESIAN_POINT ( 'NONE',  ( -45.63765681737091739, -283.4933357034532833, -342.9604870063594717 ) ) ;
#92507=CARTESIAN_POINT ( 'NONE',  ( -39.58618975457473255, -139.6688266294182768, -364.8155837051159551 ) ) ;
#92509=CARTESIAN_POINT ( 'NONE',  ( 172.5651499870576231, 243.3239573015568453, -178.9755940783880988 ) ) ;
#92510=CARTESIAN_POINT ( 'NONE',  ( -102.8603717599729350, -253.7444470676181822, -324.0947072860470826 ) ) ;
#92512=CARTESIAN_POINT ( 'NONE',  ( 20.95941956308728038, -275.3690919381396611, -314.5604524820059851 ) ) ;
#92513=CARTESIAN_POINT ( 'NONE',  ( -32.65760476330481765, -273.0328654814960032, -197.1892240351786256 ) ) ;
#92514=CARTESIAN_POINT ( 'NONE',  ( -108.3206973038857939, -295.6803290092203156, -300.1892476724093513 ) ) ;
#92515=CARTESIAN_POINT ( 'NONE',  ( -20.76932496182354271, -109.4398534507196246, -359.3069450751410159 ) ) ;
#92516=CARTESIAN_POINT ( 'NONE',  ( 25.74745274442921783, -273.6618922733635486, -227.0590612495184928 ) ) ;
#92517=CARTESIAN_POINT ( 'NONE',  ( -110.4970624660761160, -298.5762250677697693, -257.7453166657177235 ) ) ;
#92518=CARTESIAN_POINT ( 'NONE',  ( -52.44683329288052676, -292.9339375586183110, -198.5729441275987313 ) ) ;
#92520=CARTESIAN_POINT ( 'NONE',  ( -98.05527222062868020, -298.1226551495561807, -223.3645609732990920 ) ) ;
#92522=CARTESIAN_POINT ( 'NONE',  ( 33.44662823560920373, -287.8054138151556458, -252.2274694614163195 ) ) ;
#92523=CARTESIAN_POINT ( 'NONE',  ( -69.45110713615979137, -296.2668742305835963, -340.1834333749815187 ) ) ;
#92524=CARTESIAN_POINT ( 'NONE',  ( -53.27037787407919467, -295.7433601446153375, -345.6871525281212030 ) ) ;
#92525=CARTESIAN_POINT ( 'NONE',  ( 18.47521582680869656, -293.0504065899468742, -223.3135686541082805 ) ) ;
#92527=CARTESIAN_POINT ( 'NONE',  ( 29.95645263875353592, -277.0213912549139081, -236.0060189523225347 ) ) ;
#92529=CARTESIAN_POINT ( 'NONE',  ( 21.02351632912151302, -280.3824454693394728, -220.2109681438771247 ) ) ;
#92530=CARTESIAN_POINT ( 'NONE',  ( -5.215624345412746443, -275.4269267851343557, -204.5344578001107436 ) ) ;
#92531=CARTESIAN_POINT ( 'NONE',  ( 23.65289900751695740, -276.7016712331484882, -225.0440914682972107 ) ) ;
#92532=CARTESIAN_POINT ( 'NONE',  ( -92.15527082730963571, -275.8501680888918486, -322.1455895656765165 ) ) ;
#92533=CARTESIAN_POINT ( 'NONE',  ( -86.17453365271745724, -298.0045697617848646, -215.9621562474705740 ) ) ;
#92534=CARTESIAN_POINT ( 'NONE',  ( -88.92774287512330034, -294.3687337769426335, -322.9137460969129165 ) ) ;
#92536=CARTESIAN_POINT ( 'NONE',  ( -88.89486020009987044, -279.8428512276703373, -213.2489599978644605 ) ) ;
#92537=CARTESIAN_POINT ( 'NONE',  ( -53.95186679877729574, -277.4379230936123690, -341.4984353207633490 ) ) ;
#92538=CARTESIAN_POINT ( 'NONE',  ( -35.14550288652753096, -284.7639856951500974, -193.8727361304423482 ) ) ;
#92539=CARTESIAN_POINT ( 'NONE',  ( -45.94591216823866375, -299.9434374326102102, -195.6885262199777173 ) ) ;
#92541=CARTESIAN_POINT ( 'NONE',  ( 33.18765048848243282, -286.4929084700483486, -250.9134335727029566 ) ) ;
#92542=CARTESIAN_POINT ( 'NONE',  ( -1.455390797629685151, -278.7747988070152019, -205.6297745915796327 ) ) ;
#92543=CARTESIAN_POINT ( 'NONE',  ( -92.63930732343847296, -277.8145787173258441, -221.7873507051324111 ) ) ;
#92544=CARTESIAN_POINT ( 'NONE',  ( -97.09191659137582064, -282.0213189636901348, -314.7596070663852288 ) ) ;
#92545=CARTESIAN_POINT ( 'NONE',  ( -1.595886038607218005, -288.5257171740798867, -204.3704180865621254 ) ) ;
#92546=CARTESIAN_POINT ( 'NONE',  ( -3.671716595751149725, -277.8025039403691494, -335.5796944374403097 ) ) ;
#92548=CARTESIAN_POINT ( 'NONE',  ( -100.0267504248804613, -293.1090998541118893, -229.0903940957017255 ) ) ;
#92549=CARTESIAN_POINT ( 'NONE',  ( -81.96948824083577279, -275.8910997205643980, -331.8618052930501108 ) ) ;
#92550=CARTESIAN_POINT ( 'NONE',  ( 33.60610856450742290, -275.9714382879130312, -252.7457522400398204 ) ) ;
#92551=CARTESIAN_POINT ( 'NONE',  ( 30.35889149930225983, -283.1217076853852177, -237.5817215595189396 ) ) ;
#92552=CARTESIAN_POINT ( 'NONE',  ( 115.2448031289451222, -296.6656502513747569, -195.3611179825600175 ) ) ;
#92553=CARTESIAN_POINT ( 'NONE',  ( 37.25736755183265103, -289.6294585688051484, -282.6920613661519610 ) ) ;
#92554=CARTESIAN_POINT ( 'NONE',  ( -39.59235620295065416, -293.0802274217718377, -345.3399974340590006 ) ) ;
#92556=CARTESIAN_POINT ( 'NONE',  ( -59.60922381712671836, -272.4425950688236071, -200.2692765529102132 ) ) ;
#92557=CARTESIAN_POINT ( 'NONE',  ( 25.91257362791393604, -291.1639128296090462, -231.4078223145774587 ) ) ;
#92558=CARTESIAN_POINT ( 'NONE',  ( 185.2614386149834900, 255.8498544563436212, -168.8850006258623466 ) ) ;
#92560=CARTESIAN_POINT ( 'NONE',  ( -40.33115375556467086, -287.5689444528201193, -346.6221696820359170 ) ) ;
#92561=CARTESIAN_POINT ( 'NONE',  ( -108.8635532650809381, -285.9147292358250638, -288.5563080322319820 ) ) ;
#92562=CARTESIAN_POINT ( 'NONE',  ( 34.11183131551798198, -286.1246203789885385, -296.3668695348035271 ) ) ;
#92563=CARTESIAN_POINT ( 'NONE',  ( -109.5103547139871267, -286.1657300977041700, -255.9715309889180048 ) ) ;
#92564=CARTESIAN_POINT ( 'NONE',  ( -106.6886409418972761, -285.6658981906218742, -246.8871124019647141 ) ) ;
#92565=CARTESIAN_POINT ( 'NONE',  ( -36.42427561246834244, -294.0434887318140795, -194.9987451145523494 ) ) ;
#92566=CARTESIAN_POINT ( 'NONE',  ( 38.19202618707399211, -273.6066014436967180, -268.3685356935095001 ) ) ;
#92568=CARTESIAN_POINT ( 'NONE',  ( 21.71713412213653882, -276.5500505333026808, -319.7351839345006397 ) ) ;
#92570=CARTESIAN_POINT ( 'NONE',  ( -87.67176597078768907, -289.4354698685853009, -214.0033441812990986 ) ) ;
#92571=CARTESIAN_POINT ( 'NONE',  ( -2.725110648043647110, -276.6072517076405006, -339.1558201891682529 ) ) ;
#92572=CARTESIAN_POINT ( 'NONE',  ( -111.3707607570620439, -298.6605334229448090, -260.4017289942382263 ) ) ;
#92575=CARTESIAN_POINT ( 'NONE',  ( -109.1431343510291185, -283.4431751508562911, -254.6244932806141605 ) ) ;
#92577=CARTESIAN_POINT ( 'NONE',  ( -33.97878292851464721, -278.0943049767492994, -195.4365463201227726 ) ) ;
#92579=CARTESIAN_POINT ( 'NONE',  ( 21.33028221965052751, -273.3699046859019859, -221.5727357356213076 ) ) ;
#92580=CARTESIAN_POINT ( 'NONE',  ( -95.35897416353009248, -277.2759307164053553, -314.8345772815358714 ) ) ;
#92582=CARTESIAN_POINT ( 'NONE',  ( -38.33237814269151755, -296.5849167835328899, -344.0477946042022950 ) ) ;
#92583=CARTESIAN_POINT ( 'NONE',  ( 38.49119835734698825, -280.3245098778544389, -258.5767065696824716 ) ) ;
#92584=CARTESIAN_POINT ( 'NONE',  ( -72.22613468238559165, -296.4668535342543692, -334.7686355178615827 ) ) ;
#92585=CARTESIAN_POINT ( 'NONE',  ( -110.3242968023328530, -297.5765356712250309, -293.3579071742995552 ) ) ;
#92586=CARTESIAN_POINT ( 'NONE',  ( -77.51020470942363261, -297.3301747459440207, -209.3455464253848959 ) ) ;
#92587=CARTESIAN_POINT ( 'NONE',  ( -30.65330466139904075, -294.1368928967606848, -195.6599398481674257 ) ) ;
#92588=CARTESIAN_POINT ( 'NONE',  ( -9.995946222698144368, -286.5660639713516389, -198.3236971908257544 ) ) ;
#92589=CARTESIAN_POINT ( 'NONE',  ( -49.49733294339457501, -272.0384817288738759, -195.5248500825431677 ) ) ;
#92590=CARTESIAN_POINT ( 'NONE',  ( -37.98031595921003856, -285.8776791959257935, -193.3637662465722258 ) ) ;
#92591=CARTESIAN_POINT ( 'NONE',  ( -27.36290517942728684, -282.1593308363171104, -196.3339794954778199 ) ) ;
#92593=CARTESIAN_POINT ( 'NONE',  ( -73.66194086058604285, -284.6161423653227871, -206.7521696973063570 ) ) ;
#92594=CARTESIAN_POINT ( 'NONE',  ( -59.46233846113180732, -287.3384259614666121, -342.0247629238015747 ) ) ;
#92595=CARTESIAN_POINT ( 'NONE',  ( 185.7741171649701926, 251.7621132184994508, -165.9827577097485118 ) ) ;
#92596=CARTESIAN_POINT ( 'NONE',  ( 19.56707197325058445, -286.4123357593953187, -224.5223012479260944 ) ) ;
#92597=CARTESIAN_POINT ( 'NONE',  ( 11.35262850330516926, -283.3376542625996990, -329.7736788346502976 ) ) ;
#92598=CARTESIAN_POINT ( 'NONE',  ( -110.2037608184899398, -289.9178898456356706, -246.0299938682769607 ) ) ;
#92599=CARTESIAN_POINT ( 'NONE',  ( -70.90081936161800513, -281.2168859418254101, -201.9489411800058178 ) ) ;
#92600=CARTESIAN_POINT ( 'NONE',  ( -96.44720905804928179, -280.5242289289388395, -221.7625866177410785 ) ) ;
#92601=CARTESIAN_POINT ( 'NONE',  ( 34.23025929059489414, -281.5758460622283224, -284.7925453191211886 ) ) ;
#92602=CARTESIAN_POINT ( 'NONE',  ( 10.74849234607196102, -276.7166477329472514, -212.7402473473817963 ) ) ;
#92603=CARTESIAN_POINT ( 'NONE',  ( -27.74783466667040344, -294.9336544129975550, -346.8143956828052410 ) ) ;
#92604=CARTESIAN_POINT ( 'NONE',  ( -107.5888038298831333, -288.2434894918519603, -295.6037648891197591 ) ) ;
#92605=CARTESIAN_POINT ( 'NONE',  ( -93.84304463315147871, -296.1320722921035440, -223.6315930993400514 ) ) ;
#92607=ORIENTED_EDGE ( 'NONE', *, *, #58963, .T. ) ;
#92608=CARTESIAN_POINT ( 'NONE',  ( 26.81223256635550811, -283.9820507180563709, -308.2199796537997258 ) ) ;
#92609=CARTESIAN_POINT ( 'NONE',  ( -96.42802146085365678, -295.6183382412937704, -313.2881037232178869 ) ) ;
#92610=CARTESIAN_POINT ( 'NONE',  ( 34.16958999451200896, -294.2777507999552995, -242.5083317978782134 ) ) ;
#92611=CARTESIAN_POINT ( 'NONE',  ( 5.658734947701425710, -283.1033929054121927, -329.4784187595963658 ) ) ;
#92613=CARTESIAN_POINT ( 'NONE',  ( 25.95735759923632457, -274.0357539459441796, -226.9091428178749652 ) ) ;
#92614=CARTESIAN_POINT ( 'NONE',  ( -98.07399181643657471, -290.5727831894181463, -317.5299798870772179 ) ) ;
#92615=CARTESIAN_POINT ( 'NONE',  ( -93.49979086451075716, -281.9894643474612508, -321.2387422337883436 ) ) ;
#92616=CARTESIAN_POINT ( 'NONE',  ( -108.7772606237062263, -290.5213165391426742, -299.0439523635328101 ) ) ;
#92617=CARTESIAN_POINT ( 'NONE',  ( 5.860550149236601669, -288.7817084345722947, -329.2939333119965113 ) ) ;
#92620=CARTESIAN_POINT ( 'NONE',  ( 200.9980625852972764, 289.9378660408568749, -82.33773636192533729 ) ) ;
#92621=CARTESIAN_POINT ( 'NONE',  ( -110.4542110544635705, -288.2666405000204577, -253.6410175316879361 ) ) ;
#92623=CARTESIAN_POINT ( 'NONE',  ( -92.43168022879876844, -278.1601237746265269, -221.9755070720262040 ) ) ;
#92624=CARTESIAN_POINT ( 'NONE',  ( 16.01543713708688799, -274.4508111130603538, -214.8745412785359576 ) ) ;
#92625=CARTESIAN_POINT ( 'NONE',  ( -112.2264314465326009, -280.5483375777556034, -270.6704305942496376 ) ) ;
#92626=CARTESIAN_POINT ( 'NONE',  ( 155.2251193104848710, 204.5823050655612860, -215.4134129893866998 ) ) ;
#92627=CARTESIAN_POINT ( 'NONE',  ( 38.59930615872821136, -280.0144127159293248, -261.4369446313376670 ) ) ;
#92628=CARTESIAN_POINT ( 'NONE',  ( -72.19880938486630839, -281.5357693747013172, -336.3673960131706053 ) ) ;
#92629=CARTESIAN_POINT ( 'NONE',  ( -95.71834651478569356, -297.6490401164263062, -319.0243394009386293 ) ) ;
#92630=CARTESIAN_POINT ( 'NONE',  ( 31.60020728302153614, -294.3678309350707991, -294.6994515822245262 ) ) ;
#92632=CARTESIAN_POINT ( 'NONE',  ( -82.01562743920962362, -290.1137337338688553, -211.9402093550817483 ) ) ;
#92633=CARTESIAN_POINT ( 'NONE',  ( 13.89037694804752121, -275.3997153851897224, -212.9437639542252043 ) ) ;
#92634=CARTESIAN_POINT ( 'NONE',  ( -64.56878677730624361, -273.6865639375479873, -202.6151809828252226 ) ) ;
#92642=CARTESIAN_POINT ( 'NONE',  ( 15.47257245861199237, -281.9001003777036090, -219.4469127431976574 ) ) ;
#92643=CARTESIAN_POINT ( 'NONE',  ( -95.14968307826980265, -280.9864978662519661, -221.0236730041305862 ) ) ;
#92644=CARTESIAN_POINT ( 'NONE',  ( -109.7328037496047131, -283.4608186238167491, -281.7744903052087579 ) ) ;
#92645=CARTESIAN_POINT ( 'NONE',  ( 18.88484054146146462, -282.7334872640489039, -221.8705737250467962 ) ) ;
#92646=CARTESIAN_POINT ( 'NONE',  ( 36.04268951173919788, -274.1201099776182559, -277.1019716827017874 ) ) ;
#92651=CARTESIAN_POINT ( 'NONE',  ( -67.63551481766778295, -278.2424812026052905, -340.9758729023049568 ) ) ;
#92655=CARTESIAN_POINT ( 'NONE',  ( -112.2657325385600586, -286.4291764931783746, -278.4107247322160106 ) ) ;
#92656=CARTESIAN_POINT ( 'NONE',  ( 20.31645664254551775, -292.1157217921819438, -225.3059721731350464 ) ) ;
#92657=CARTESIAN_POINT ( 'NONE',  ( 39.60034901838157140, -286.9157285095449765, -271.5579925626856266 ) ) ;
#92658=CARTESIAN_POINT ( 'NONE',  ( -72.84061110800165295, -283.8150037965478987, -205.4021040435784471 ) ) ;
#92659=CARTESIAN_POINT ( 'NONE',  ( -93.69471392446111224, -283.7935980199576989, -223.0355143973431495 ) ) ;
#92660=CARTESIAN_POINT ( 'NONE',  ( 24.34180251449186727, -286.3521244846036780, -311.2880405816613347 ) ) ;
#92661=CARTESIAN_POINT ( 'NONE',  ( 35.74624249197428583, -282.6619248833271172, -263.0968682974351509 ) ) ;
#92662=CARTESIAN_POINT ( 'NONE',  ( 10.52924183781424716, -272.7126596815619450, -212.5582384100262914 ) ) ;
#92663=CARTESIAN_POINT ( 'NONE',  ( -111.5757103880138459, -283.1693687970175688, -253.1636722546211615 ) ) ;
#92664=CARTESIAN_POINT ( 'NONE',  ( -56.89354169956914831, -299.8003121456598592, -197.9005983948055416 ) ) ;
#92665=CARTESIAN_POINT ( 'NONE',  ( -79.87921786420695014, -283.4785847636560447, -208.3258274069511060 ) ) ;
#92666=CARTESIAN_POINT ( 'NONE',  ( -81.43908271641872432, -280.3770999615201731, -211.8266766385823132 ) ) ;
#92667=CARTESIAN_POINT ( 'NONE',  ( 34.09843068951497713, -289.2491378171986867, -246.8209998709012609 ) ) ;
#92670=CARTESIAN_POINT ( 'NONE',  ( 10.19353815006491715, -294.6215679275500179, -211.5595428712367720 ) ) ;
#92673=CARTESIAN_POINT ( 'NONE',  ( -108.1609338607598403, -276.2304972267014591, -295.2096012446178861 ) ) ;
#92674=CARTESIAN_POINT ( 'NONE',  ( -113.8450395044615959, -289.8460501988727174, -262.6429917538795848 ) ) ;
#92675=CARTESIAN_POINT ( 'NONE',  ( -68.87749863574900644, -293.8736536370661270, -337.0978145567249271 ) ) ;
#92676=CARTESIAN_POINT ( 'NONE',  ( -92.56802169174439143, -277.9246592105881746, -221.8518060719377161 ) ) ;
#92677=CARTESIAN_POINT ( 'NONE',  ( -34.39520772895804868, -296.2290015565217232, -196.1268563079971727 ) ) ;
#92678=CARTESIAN_POINT ( 'NONE',  ( -57.80822982711061542, -293.0975594957903354, -199.7220131558359242 ) ) ;
#92679=CARTESIAN_POINT ( 'NONE',  ( -95.95921662488163406, -286.4090924074130839, -317.1477375740089997 ) ) ;
#92680=CARTESIAN_POINT ( 'NONE',  ( -112.7017298340046381, -295.1842929837864631, -258.2962494915011575 ) ) ;
#92681=CARTESIAN_POINT ( 'NONE',  ( 20.14938420122146923, -289.7993748913999070, -316.6343893207871929 ) ) ;
#92682=CARTESIAN_POINT ( 'NONE',  ( -61.34692068096671846, -289.9845997026833402, -198.2104676535045371 ) ) ;
#92684=CARTESIAN_POINT ( 'NONE',  ( -107.9658625752614114, -292.2493396486327129, -249.6377814691441301 ) ) ;
#92686=CARTESIAN_POINT ( 'NONE',  ( -20.04387780123211371, -293.0828868104173921, -199.2215553212956536 ) ) ;
#92688=CARTESIAN_POINT ( 'NONE',  ( -106.9063117174093378, -292.1710781583050220, -238.1601826525033516 ) ) ;
#92689=CARTESIAN_POINT ( 'NONE',  ( 37.77418962071515551, -279.4955715038523749, -264.3602923769542485 ) ) ;
#92690=CARTESIAN_POINT ( 'NONE',  ( -25.40909225615754252, -292.2083475194318112, -198.2914966976853464 ) ) ;
#92691=CARTESIAN_POINT ( 'NONE',  ( -16.99199079425166303, -280.3078913178703715, -196.0988171157767113 ) ) ;
#92692=CARTESIAN_POINT ( 'NONE',  ( 13.66360259252715359, -282.0274083300692496, -328.0879720463673266 ) ) ;
#92693=CARTESIAN_POINT ( 'NONE',  ( 30.01301615046398652, -285.9869643770724110, -303.3511595203857496 ) ) ;
#92694=CARTESIAN_POINT ( 'NONE',  ( 32.50892429892402902, -280.0226914016827777, -295.6477215796933251 ) ) ;
#92695=CARTESIAN_POINT ( 'NONE',  ( -65.11249984092846432, -283.6891656544832472, -200.6782345273111332 ) ) ;
#92697=CARTESIAN_POINT ( 'NONE',  ( -61.80684417870997294, -278.2198669557403150, -198.0270152615564712 ) ) ;
#92698=CARTESIAN_POINT ( 'NONE',  ( 11.88971723974640682, -285.6377477441452015, -211.4890898157504751 ) ) ;
#92699=CARTESIAN_POINT ( 'NONE',  ( 23.18017701616185278, -275.7843138273685213, -229.2326404529472939 ) ) ;
#92701=CARTESIAN_POINT ( 'NONE',  ( 21.62081414357954756, -294.5357465397808596, -225.9779868656659119 ) ) ;
#92702=CARTESIAN_POINT ( 'NONE',  ( 11.39579676911217554, -276.1375412612125047, -211.4428845380559778 ) ) ;
#92703=CARTESIAN_POINT ( 'NONE',  ( -68.05017661106406024, -277.1335245801039378, -336.6249791158144262 ) ) ;
#92704=CARTESIAN_POINT ( 'NONE',  ( -114.1879726621797317, -290.7796524376174716, -265.4979500743418157 ) ) ;
#92705=CONICAL_SURFACE ( 'NONE', #30741, 2.888540232138026020, 0.09862129276974965220 ) ;
#92706=CARTESIAN_POINT ( 'NONE',  ( 0.6710972074730073844, -278.6342487142701998, -204.9996133326930590 ) ) ;
#92707=CARTESIAN_POINT ( 'NONE',  ( -69.10885461959507836, -290.6825606475176755, -204.3604820173550252 ) ) ;
#92710=CARTESIAN_POINT ( 'NONE',  ( -25.25587232342336819, -292.8980477486874747, -344.4335943646663623 ) ) ;
#92714=CARTESIAN_POINT ( 'NONE',  ( 4.544050151169820140, -292.1418306738939350, -210.4361500949838160 ) ) ;
#92716=CARTESIAN_POINT ( 'NONE',  ( 34.45848030099739390, -273.0523547857346784, -270.3937649182068412 ) ) ;
#92717=CARTESIAN_POINT ( 'NONE',  ( -113.7103600977389561, -295.5132081979551231, -278.1487997306520015 ) ) ;
#92718=CARTESIAN_POINT ( 'NONE',  ( -92.06920271828326463, -285.1291852741715616, -323.8232422630305791 ) ) ;
#92719=CARTESIAN_POINT ( 'NONE',  ( 35.55278243395914473, -287.3225164958134314, -265.5888179833442564 ) ) ;
#92720=CARTESIAN_POINT ( 'NONE',  ( 34.50543289770274669, -276.8574090467004680, -253.9127791127628768 ) ) ;
#92721=CARTESIAN_POINT ( 'NONE',  ( -111.3640211395889139, -294.7013876501425784, -260.3517381561532034 ) ) ;
#92722=CARTESIAN_POINT ( 'NONE',  ( -111.3885459438542824, -298.3334891209181592, -268.7326610350772853 ) ) ;
#92723=CARTESIAN_POINT ( 'NONE',  ( 28.37925123826012808, -274.7891584195456858, -303.1541860474146688 ) ) ;
#92725=CARTESIAN_POINT ( 'NONE',  ( -111.6005434785387536, -296.4752008878752463, -249.8819710408546939 ) ) ;
#92726=CARTESIAN_POINT ( 'NONE',  ( 4.442736434292411829, -290.4042467313579436, -332.0299016112302866 ) ) ;
#92727=CARTESIAN_POINT ( 'NONE',  ( -28.85729229363806780, -296.1582027931529524, -195.3640018882764195 ) ) ;
#92729=CARTESIAN_POINT ( 'NONE',  ( -34.56583242676096290, -289.6679083174312268, -343.4599794784073197 ) ) ;
#92731=CARTESIAN_POINT ( 'NONE',  ( -3.749715823618728461, -279.5433076938443833, -201.3220181983409418 ) ) ;
#92732=CARTESIAN_POINT ( 'NONE',  ( -95.49945937741655655, -297.8847213535917717, -219.9727116720819993 ) ) ;
#92733=CARTESIAN_POINT ( 'NONE',  ( -109.6109264662099463, -288.3992524881264785, -293.2805329165127546 ) ) ;
#92734=CARTESIAN_POINT ( 'NONE',  ( -112.2842387552876176, -296.6646875703952446, -288.0067575520780565 ) ) ;
#92735=CARTESIAN_POINT ( 'NONE',  ( 21.00813975319014659, -293.2691042099392575, -226.4591399783664372 ) ) ;
#92740=CARTESIAN_POINT ( 'NONE',  ( 35.72713028738823482, -289.3513168716552855, -292.3986689058187380 ) ) ;
#92741=CARTESIAN_POINT ( 'NONE',  ( -19.11405058567862625, -276.7662352645559167, -190.3538533559490702 ) ) ;
#92743=CARTESIAN_POINT ( 'NONE',  ( 35.23424366332909585, -280.5779367435727636, -244.7846100892792265 ) ) ;
#92744=CARTESIAN_POINT ( 'NONE',  ( -93.01229214289865865, -285.8538830925358525, -320.3885274131033043 ) ) ;
#92745=CARTESIAN_POINT ( 'NONE',  ( 39.05135671310836898, -286.1061451333618493, -268.7157737124992423 ) ) ;
#92746=CARTESIAN_POINT ( 'NONE',  ( -79.00013505429254224, -287.6980962825746246, -332.1150732710872830 ) ) ;
#92747=CARTESIAN_POINT ( 'NONE',  ( 34.55025634783915933, -277.1047257664152994, -246.2824693394957194 ) ) ;
#92751=CARTESIAN_POINT ( 'NONE',  ( -97.64882855119962812, -277.9798621266210148, -311.4956565281365215 ) ) ;
#92752=CARTESIAN_POINT ( 'NONE',  ( -39.69621630988346084, -279.3704233127705265, -197.2845749876478578 ) ) ;
#92753=CARTESIAN_POINT ( 'NONE',  ( 31.58353368740714373, -277.0666814910394464, -304.1095602022843423 ) ) ;
#92754=CARTESIAN_POINT ( 'NONE',  ( -104.4383647096886705, -277.8282942715412673, -233.4010541350342862 ) ) ;
#92755=CARTESIAN_POINT ( 'NONE',  ( -104.2745392939568347, -253.7788420816588371, -324.7530620101808836 ) ) ;
#92756=CARTESIAN_POINT ( 'NONE',  ( -78.72482614818748914, -274.4503635723456227, -205.7062102539960051 ) ) ;
#92758=CARTESIAN_POINT ( 'NONE',  ( 75.28772777193687205, -300.8615142928297246, -193.9236106809661919 ) ) ;
#92759=CARTESIAN_POINT ( 'NONE',  ( -4.829096099716510437, -288.9805209788416391, -202.7746430608542312 ) ) ;
#92760=CARTESIAN_POINT ( 'NONE',  ( 82.61715650332634198, -302.0474575487106677, -194.9843264058633849 ) ) ;
#92761=CARTESIAN_POINT ( 'NONE',  ( 26.63043373960363525, -288.1429156043636794, -234.4551642000964478 ) ) ;
#92762=CARTESIAN_POINT ( 'NONE',  ( -112.4887677409936373, -286.4594547617298304, -258.7488280938900971 ) ) ;
#92763=CARTESIAN_POINT ( 'NONE',  ( 31.93984256809328315, -286.5913410514270367, -247.0381569831579043 ) ) ;
#92764=CARTESIAN_POINT ( 'NONE',  ( -111.8169800973878978, -283.8173155669605876, -289.7255276703332356 ) ) ;
#92765=CARTESIAN_POINT ( 'NONE',  ( 7.645952984501175997, -279.0773445473428183, -211.7938697157454726 ) ) ;
#92766=CARTESIAN_POINT ( 'NONE',  ( -35.93339486472894606, -287.9304181423797786, -196.1392737618143087 ) ) ;
#92767=CARTESIAN_POINT ( 'NONE',  ( 15.77240783317803619, -279.3007262354486215, -219.2039608641025268 ) ) ;
#92768=CARTESIAN_POINT ( 'NONE',  ( -69.45185937936612675, -278.7989468334097296, -336.4823929597917527 ) ) ;
#92769=CARTESIAN_POINT ( 'NONE',  ( -4.082266448267762193, -274.9953844965841654, -205.2947985567448370 ) ) ;
#92770=CARTESIAN_POINT ( 'NONE',  ( -67.90959968146094639, -288.2395223493836056, -340.6007950629511356 ) ) ;
#92771=CARTESIAN_POINT ( 'NONE',  ( 15.64958087279715038, -283.1276838130997362, -326.0035744167684584 ) ) ;
#92772=CARTESIAN_POINT ( 'NONE',  ( -109.9212842186116319, -285.3668021540639188, -244.8320977037900548 ) ) ;
#92773=CARTESIAN_POINT ( 'NONE',  ( 18.49572707474300159, -282.3870067893979581, -317.4037272379866863 ) ) ;
#92774=ORIENTED_EDGE ( 'NONE', *, *, #75186, .T. ) ;
#92777=CARTESIAN_POINT ( 'NONE',  ( -23.51374020987026725, -290.7377699108475326, -344.9066014553536093 ) ) ;
#92778=CARTESIAN_POINT ( 'NONE',  ( -11.30522686547490885, -291.0691197055824091, -198.3651785395221623 ) ) ;
#92779=CARTESIAN_POINT ( 'NONE',  ( -90.35869808522477342, -272.3373592992242038, -219.8194490478255148 ) ) ;
#92780=CARTESIAN_POINT ( 'NONE',  ( 38.22660939108778422, -292.7224300935576480, -256.1223194633552112 ) ) ;
#92781=CARTESIAN_POINT ( 'NONE',  ( -82.99076951297975313, -288.1699095240115867, -328.2132589522969965 ) ) ;
#92782=CARTESIAN_POINT ( 'NONE',  ( 25.27272622487605247, -292.3308470801798080, -309.9213489643938715 ) ) ;
#92783=CARTESIAN_POINT ( 'NONE',  ( 19.83240214985690031, -289.4043862012323416, -316.3855955452976332 ) ) ;
#92784=CARTESIAN_POINT ( 'NONE',  ( 39.58706461736021254, -296.0519495502702512, -270.3284710469133074 ) ) ;
#92786=CARTESIAN_POINT ( 'NONE',  ( -99.02093906268960666, -291.9737445061645644, -313.0304528031829818 ) ) ;
#92787=CARTESIAN_POINT ( 'NONE',  ( -111.5541497753442854, -288.3990361921856334, -282.3001608637193272 ) ) ;
#92788=CARTESIAN_POINT ( 'NONE',  ( -110.8914229348953597, -292.3630273195871041, -285.1029486988791746 ) ) ;
#92789=CARTESIAN_POINT ( 'NONE',  ( -8.172210052900707566, -287.3850792342683462, -203.1856068390513883 ) ) ;
#92790=CARTESIAN_POINT ( 'NONE',  ( 34.52645792512056744, -295.2690317622800649, -248.3384867775273221 ) ) ;
#92791=CARTESIAN_POINT ( 'NONE',  ( -113.1481451663846372, -270.7100043341520745, -270.3376630279467463 ) ) ;
#92794=CARTESIAN_POINT ( 'NONE',  ( 32.18599689650407925, -277.1528831882408213, -241.1695116136054082 ) ) ;
#92795=CARTESIAN_POINT ( 'NONE',  ( -40.33910760393814599, -281.0896855089778228, -345.3012020471741153 ) ) ;
#92796=CARTESIAN_POINT ( 'NONE',  ( -111.4635745307208481, -296.0057253443188188, -249.9135207091414657 ) ) ;
#92797=CARTESIAN_POINT ( 'NONE',  ( -24.39747877565732637, -272.4593499031792021, -197.4361741901698224 ) ) ;
#92798=CARTESIAN_POINT ( 'NONE',  ( -110.7094331762306183, -276.4681587035067309, -283.0258827709869252 ) ) ;
#92799=CARTESIAN_POINT ( 'NONE',  ( -99.62549899168176637, -274.2902654152014179, -231.5299590561883178 ) ) ;
#92802=CARTESIAN_POINT ( 'NONE',  ( -82.70891359407991672, -297.1111712945385079, -328.3673454429822982 ) ) ;
#92804=CARTESIAN_POINT ( 'NONE',  ( -102.6811405173542369, -297.8020784537931718, -237.3338632265739250 ) ) ;
#92806=CARTESIAN_POINT ( 'NONE',  ( 19.07251357880367948, -284.8800978417655756, -220.3256434277620883 ) ) ;
#92807=CARTESIAN_POINT ( 'NONE',  ( -109.1293176453904721, -272.5638151817186667, -256.8416908511349561 ) ) ;
#92809=CARTESIAN_POINT ( 'NONE',  ( -7.343129295381475075, -286.4346928648794233, -199.3884152920370525 ) ) ;
#92810=CARTESIAN_POINT ( 'NONE',  ( 18.33913858318828005, -286.4911293135903065, -217.1298548559292954 ) ) ;
#92811=CARTESIAN_POINT ( 'NONE',  ( -72.53538336964163591, -299.5689175071598243, -203.6716065847124355 ) ) ;
#92812=CARTESIAN_POINT ( 'NONE',  ( -4.765896197686079638, -292.6219760243730548, -337.7462264828085949 ) ) ;
#92814=CARTESIAN_POINT ( 'NONE',  ( -5.002626537620225911, -279.6643596081917735, -200.6593020770489204 ) ) ;
#92816=CARTESIAN_POINT ( 'NONE',  ( -114.2704648735229114, -282.0523547857346216, -270.3284710469133074 ) ) ;
#92818=CARTESIAN_POINT ( 'NONE',  ( -29.14392665854766307, -287.7408694713238901, -343.2989477736718982 ) ) ;
#92820=CARTESIAN_POINT ( 'NONE',  ( -42.83515596486595456, -287.1211847443145757, -345.2116553274981925 ) ) ;
#92821=CARTESIAN_POINT ( 'NONE',  ( -60.78917333951024204, -299.3430539754077699, -200.3309442646652485 ) ) ;
#92822=CARTESIAN_POINT ( 'NONE',  ( 14.74629461529344887, -282.1936574969902836, -214.3831060242029309 ) ) ;
#92823=CARTESIAN_POINT ( 'NONE',  ( -89.59019870554278953, -293.8039212067739072, -324.7330857885210662 ) ) ;
#92824=CARTESIAN_POINT ( 'NONE',  ( -4.827162856289269222, -282.6115206781774418, -335.7201637681377520 ) ) ;
#92825=CARTESIAN_POINT ( 'NONE',  ( -112.8890979635703644, -296.9058484947580610, -255.4073796362336566 ) ) ;
#92826=CARTESIAN_POINT ( 'NONE',  ( -84.53354290713501484, -298.9089797542448537, -213.6937905886628926 ) ) ;
#92827=CARTESIAN_POINT ( 'NONE',  ( 37.62160898672623688, -283.5824370682346967, -272.7069509557205720 ) ) ;
#92828=CARTESIAN_POINT ( 'NONE',  ( -95.79936664164830518, -294.9929660865950041, -314.4965136002880968 ) ) ;
#92831=CARTESIAN_POINT ( 'NONE',  ( 20.64539316579068995, -284.1826044300177614, -317.3849305712267324 ) ) ;
#92832=CARTESIAN_POINT ( 'NONE',  ( 104.1717476309105166, -299.5541904835127980, -192.9651424135224715 ) ) ;
#92833=CARTESIAN_POINT ( 'NONE',  ( 21.27581636871891391, -285.6952119285919025, -317.1477375740089997 ) ) ;
#92834=CARTESIAN_POINT ( 'NONE',  ( 39.39372618803411541, -274.6879006864496660, -265.4602870448940735 ) ) ;
#92835=CARTESIAN_POINT ( 'NONE',  ( 31.80172097998576319, -293.0725072112369958, -246.7903474453153763 ) ) ;
#92836=CARTESIAN_POINT ( 'NONE',  ( 36.21068992604088521, -283.0127505857650476, -265.8054985685174074 ) ) ;
#92837=CARTESIAN_POINT ( 'NONE',  ( 34.60920556017164529, -276.9374025108861019, -253.8880014605112763 ) ) ;
#92838=CARTESIAN_POINT ( 'NONE',  ( -38.70370545048507438, -284.4941871834200242, -346.7597517165867771 ) ) ;
#92839=CARTESIAN_POINT ( 'NONE',  ( 35.09296335587882254, -280.5025075061399207, -282.2080598349747333 ) ) ;
#92840=CARTESIAN_POINT ( 'NONE',  ( -106.2904436542752649, -280.9382004337196008, -240.8471990272735468 ) ) ;
#92841=CARTESIAN_POINT ( 'NONE',  ( -78.84334023757111254, -273.6759164488199758, -205.5027039353578573 ) ) ;
#92842=CARTESIAN_POINT ( 'NONE',  ( 22.63966541114735165, -276.0327784411712742, -318.6648456798098437 ) ) ;
#92843=CARTESIAN_POINT ( 'NONE',  ( 22.12979309200113320, -294.8557204715738749, -225.5899699650828722 ) ) ;
#92846=CARTESIAN_POINT ( 'NONE',  ( -98.90385110540442781, -295.2865493959877767, -226.1977049698182896 ) ) ;
#92847=CARTESIAN_POINT ( 'NONE',  ( 35.08233664242854388, -274.9328666446943430, -260.7305759664939160 ) ) ;
#92849=CARTESIAN_POINT ( 'NONE',  ( 28.98171758952452137, -295.5679498969847714, -308.2026640136495530 ) ) ;
#92850=CARTESIAN_POINT ( 'NONE',  ( -13.88894752603242999, -295.9594982902865468, -343.2855796754116113 ) ) ;
#92851=CARTESIAN_POINT ( 'NONE',  ( 33.13433877471279487, -289.8791274025601297, -295.5237165324286366 ) ) ;
#92852=CARTESIAN_POINT ( 'NONE',  ( -70.07579912940701661, -275.4841491643225595, -337.6694883478669453 ) ) ;
#92854=CARTESIAN_POINT ( 'NONE',  ( -88.05911419239056670, -279.6886364666779059, -324.8501820822274340 ) ) ;
#92855=CARTESIAN_POINT ( 'NONE',  ( -48.02337380076793494, -293.2687780946819771, -344.0830528402298114 ) ) ;
#92856=CARTESIAN_POINT ( 'NONE',  ( 12.16684849994686246, -282.5929109843434048, -213.0094912340223914 ) ) ;
#92857=CARTESIAN_POINT ( 'NONE',  ( -49.45914084493316665, -284.8144938107437838, -198.0086857638848699 ) ) ;
#92858=CARTESIAN_POINT ( 'NONE',  ( 181.7997601335249556, 252.1859019497369445, -165.9525674339327850 ) ) ;
#92860=CARTESIAN_POINT ( 'NONE',  ( -49.42084836320960051, -285.5607638911498611, -198.2944561798227596 ) ) ;
#92862=CARTESIAN_POINT ( 'NONE',  ( 37.94859159815776195, -282.4486168879772094, -255.7712419592744766 ) ) ;
#92864=CARTESIAN_POINT ( 'NONE',  ( -111.8366280341288217, -283.1220266745824574, -288.2636631830587248 ) ) ;
#92866=CARTESIAN_POINT ( 'NONE',  ( -112.1750488634762775, -279.7080529226809631, -253.2500066417094899 ) ) ;
#92867=CARTESIAN_POINT ( 'NONE',  ( -111.4967616055142514, -279.8445091054852014, -288.4084171103550034 ) ) ;
#92868=CARTESIAN_POINT ( 'NONE',  ( -53.28691492658256834, -297.7662352645559167, -340.3683826091709079 ) ) ;
#92869=CARTESIAN_POINT ( 'NONE',  ( 85.57369694988886977, 82.79219029714946032, -302.3637402596039010 ) ) ;
#92871=CARTESIAN_POINT ( 'NONE',  ( -51.94351526458655144, -275.8651589396186523, -196.9130963471600069 ) ) ;
#92872=CARTESIAN_POINT ( 'NONE',  ( -90.47616956950605527, -230.2765260023237204, -347.7368331188681623 ) ) ;
#92873=AXIS2_PLACEMENT_3D ( 'NONE', #38387, #25578, #12316 ) ;
#92874=CARTESIAN_POINT ( 'NONE',  ( -8.591038903044097452, -278.4504038211729835, -201.4753699399532820 ) ) ;
#92875=CARTESIAN_POINT ( 'NONE',  ( -76.66431668589918047, -293.2940619400229707, -205.2796147166539811 ) ) ;
#92876=CARTESIAN_POINT ( 'NONE',  ( 33.87284088849880703, -293.1188054656516329, -286.9202305669654152 ) ) ;
#92877=CARTESIAN_POINT ( 'NONE',  ( -93.55212778230500703, -289.3421493711076664, -322.9727977038713220 ) ) ;
#92879=CARTESIAN_POINT ( 'NONE',  ( -16.68376090604201778, -293.3652342773754640, -343.9812407148490934 ) ) ;
#92880=CARTESIAN_POINT ( 'NONE',  ( -16.93128338593110627, -284.7198704381099787, -199.3862139363613437 ) ) ;
#92881=CARTESIAN_POINT ( 'NONE',  ( -9.282195404500859226, -294.2831771746835443, -201.5784922947043185 ) ) ;
#92882=CARTESIAN_POINT ( 'NONE',  ( -19.63065460626670244, -284.7639404852479288, -198.8277228649770336 ) ) ;
#92883=CARTESIAN_POINT ( 'NONE',  ( 18.88237579884572170, -283.5353150190501879, -317.7103196935150322 ) ) ;
#92885=CARTESIAN_POINT ( 'NONE',  ( -103.0207607332826996, -292.0147752144574724, -230.5209505443164630 ) ) ;
#92886=CARTESIAN_POINT ( 'NONE',  ( 26.50958233963024568, -281.5593876900824739, -234.8505256370674772 ) ) ;
#92887=CARTESIAN_POINT ( 'NONE',  ( 15.19515410428097368, -293.1248168212677001, -326.1095499348656404 ) ) ;
#92888=AXIS2_PLACEMENT_3D ( 'NONE', #27049, #54513, #48340 ) ;
#92889=CARTESIAN_POINT ( 'NONE',  ( 36.63174046260067485, -288.6165656147635445, -291.1961425369566427 ) ) ;
#92891=CARTESIAN_POINT ( 'NONE',  ( -37.49516900964340493, -289.5463332417454012, -347.3124881977668679 ) ) ;
#92892=CARTESIAN_POINT ( 'NONE',  ( 17.82692498352302835, -288.4008067648674114, -318.2429006435521615 ) ) ;
#92893=VERTEX_POINT ( 'NONE', #34877 ) ;
#92895=CARTESIAN_POINT ( 'NONE',  ( -36.26780400159414341, -296.8992701365683047, -346.1312037958138035 ) ) ;
#92896=CARTESIAN_POINT ( 'NONE',  ( -70.50006269974683448, -296.3089134298974727, -201.4131574120132200 ) ) ;
#92897=CARTESIAN_POINT ( 'NONE',  ( -91.14884666236504529, -276.8990072520734884, -320.1158736413113388 ) ) ;
#92898=CARTESIAN_POINT ( 'NONE',  ( -76.39607400263459169, -273.0525669962132156, -204.0101741712486216 ) ) ;
#92899=CARTESIAN_POINT ( 'NONE',  ( -10.25298149166816764, -293.1719150093079520, -338.8951173952573868 ) ) ;
#92900=CARTESIAN_POINT ( 'NONE',  ( 34.88703270323007644, -277.5232384338306133, -286.5738290956944070 ) ) ;
#92901=CARTESIAN_POINT ( 'NONE',  ( -101.7783570804827065, -271.1896539146687246, -233.3961333614975899 ) ) ;
#92902=CARTESIAN_POINT ( 'NONE',  ( -2.944157319955445384, -295.7919262268183047, -335.1989121650426569 ) ) ;
#92903=CARTESIAN_POINT ( 'NONE',  ( -82.53962862501616371, -296.7656260072712371, -328.1438806329443878 ) ) ;
#92904=CARTESIAN_POINT ( 'NONE',  ( -25.01691449717860394, -296.4977570206539781, -345.6113000395394010 ) ) ;
#92905=CARTESIAN_POINT ( 'NONE',  ( -112.4046897001549041, -294.4900537445482200, -275.1954604732495682 ) ) ;
#92906=CARTESIAN_POINT ( 'NONE',  ( -31.92679025380941482, -298.7696888616834485, -193.4624692755411388 ) ) ;
#92907=CARTESIAN_POINT ( 'NONE',  ( -79.85644511805752188, -290.0396288688492632, -210.2331097033479352 ) ) ;
#92908=CARTESIAN_POINT ( 'NONE',  ( -103.8145530635746496, -275.0136687216667042, -235.5158606163035131 ) ) ;
#92909=CARTESIAN_POINT ( 'NONE',  ( -49.71552673843546444, -274.3908660882439676, -194.3704383794815271 ) ) ;
#92910=CARTESIAN_POINT ( 'NONE',  ( -108.9045957971519698, -296.6931218976637865, -284.9436818444152664 ) ) ;
#92911=CARTESIAN_POINT ( 'NONE',  ( 27.85071668681591106, -283.0298027938352448, -232.5675260595379825 ) ) ;
#92912=CARTESIAN_POINT ( 'NONE',  ( 33.10525203171939523, -280.6207722733769288, -300.3380091289097891 ) ) ;
#92913=CARTESIAN_POINT ( 'NONE',  ( -30.23258465161730157, -282.3130283196431947, -346.9298665922988789 ) ) ;
#92914=CARTESIAN_POINT ( 'NONE',  ( 39.21666439910256230, -274.8035345910203091, -262.5988920357814891 ) ) ;
#92915=CARTESIAN_POINT ( 'NONE',  ( -2.735067194011227887, -278.9017805312781775, -202.4582409639698710 ) ) ;
#92916=CARTESIAN_POINT ( 'NONE',  ( -95.38508574367567405, -277.2094317739892517, -222.5813593959834691 ) ) ;
#92917=CARTESIAN_POINT ( 'NONE',  ( 3.270126175024986370, -273.1840322527841067, -208.9320209849939545 ) ) ;
#92918=CARTESIAN_POINT ( 'NONE',  ( 32.90753917720181221, -277.8951031929577198, -296.7759385152284608 ) ) ;
#92921=CARTESIAN_POINT ( 'NONE',  ( -55.84550241976100438, -293.5270836603111775, -344.0603941803383350 ) ) ;
#92922=CARTESIAN_POINT ( 'NONE',  ( -53.02191043809781945, -289.8723591186568456, -196.6020361752016470 ) ) ;
#92923=CARTESIAN_POINT ( 'NONE',  ( -7.190202469943082875, -292.4368558564719933, -199.4956340707202287 ) ) ;
#92924=CARTESIAN_POINT ( 'NONE',  ( -20.51121980868179051, -278.8368119763187565, -343.6727349932750144 ) ) ;
#92925=CARTESIAN_POINT ( 'NONE',  ( -16.04911868242266948, -272.3271897846799448, -198.3929367641325143 ) ) ;
#92928=CARTESIAN_POINT ( 'NONE',  ( -16.51482975628218597, -284.7053831647747870, -343.0483961740949326 ) ) ;
#92930=CARTESIAN_POINT ( 'NONE',  ( -55.16793606341359890, -283.8228492554528657, -197.4575361682418588 ) ) ;
#92932=CARTESIAN_POINT ( 'NONE',  ( 29.84741888892822814, -292.7423746513612741, -299.9035076864358302 ) ) ;
#92933=CARTESIAN_POINT ( 'NONE',  ( 36.89010749396630473, -285.7009403480349761, -271.0711986815784940 ) ) ;
#92935=CARTESIAN_POINT ( 'NONE',  ( -39.77886561469352245, -293.0825783057031799, -345.3342840592745802 ) ) ;
#92936=CARTESIAN_POINT ( 'NONE',  ( -109.5746610762987814, -282.7192859744682778, -294.9600428515508952 ) ) ;
#92937=CARTESIAN_POINT ( 'NONE',  ( -65.13610088866967374, -281.2829201111977113, -201.9951052112525360 ) ) ;
#92938=CARTESIAN_POINT ( 'NONE',  ( -49.29797004043021502, -287.1082131275349525, -194.6435561421023124 ) ) ;
#92939=CARTESIAN_POINT ( 'NONE',  ( 25.45599057564264811, -279.2191912456597152, -227.4858155928311305 ) ) ;
#92940=CARTESIAN_POINT ( 'NONE',  ( 27.03046584175159950, -288.0227341230162210, -304.8957891121283978 ) ) ;
#92942=CARTESIAN_POINT ( 'NONE',  ( -68.26866413860632576, -278.8917934645388073, -337.1499535678766506 ) ) ;
#92943=CARTESIAN_POINT ( 'NONE',  ( -91.07952257907312799, -278.6428103739348217, -320.0820335829324677 ) ) ;
#92944=CARTESIAN_POINT ( 'NONE',  ( -65.29124487541788824, -287.6685758785660596, -200.3670538258703573 ) ) ;
#92946=CARTESIAN_POINT ( 'NONE',  ( -31.90740253627349077, -297.9517514386424182, -193.3612665261361485 ) ) ;
#92947=CARTESIAN_POINT ( 'NONE',  ( 37.32495697097782283, -289.5047005553334998, -268.2411436631842889 ) ) ;
#92949=CARTESIAN_POINT ( 'NONE',  ( -19.11405058567862625, -276.7662352645559167, -190.3538533559490702 ) ) ;
#92951=CARTESIAN_POINT ( 'NONE',  ( -16.26637843760867597, -272.3236647173372376, -198.1554498022277642 ) ) ;
#92952=CARTESIAN_POINT ( 'NONE',  ( 25.04781221936262270, -292.5368937865397356, -314.1330434568142209 ) ) ;
#92953=CARTESIAN_POINT ( 'NONE',  ( -91.88666206080398524, -296.7543274982097614, -221.7521109003415631 ) ) ;
#92954=CARTESIAN_POINT ( 'NONE',  ( 5.109105701991394355, -288.1575443531618816, -210.0605157465149944 ) ) ;
#92956=CARTESIAN_POINT ( 'NONE',  ( 33.20391960337276060, -283.6070405065344175, -292.9176950231448018 ) ) ;
#92957=CARTESIAN_POINT ( 'NONE',  ( -59.83636354609197383, -290.7633070791865180, -343.3857467687143981 ) ) ;
#92958=CARTESIAN_POINT ( 'NONE',  ( -69.13698276741453697, -290.7768347648495819, -339.9625028512141967 ) ) ;
#92959=CARTESIAN_POINT ( 'NONE',  ( -92.18709541518154538, -285.8362080841440616, -321.5175766653520100 ) ) ;
#92960=CARTESIAN_POINT ( 'NONE',  ( -111.4399386335719129, -278.4564002010822037, -291.3003408645210470 ) ) ;
#92961=CARTESIAN_POINT ( 'NONE',  ( 33.10004141577986303, -291.9849371363591217, -297.6974535867205987 ) ) ;
#92962=CARTESIAN_POINT ( 'NONE',  ( -2.388245089953710654, -280.3349970199848258, -201.7369448303928152 ) ) ;
#92964=CARTESIAN_POINT ( 'NONE',  ( -29.88902839056538951, -276.0079089227348845, -196.5009584666116780 ) ) ;
#92965=CARTESIAN_POINT ( 'NONE',  ( 39.58706461736021254, -296.0519495502702512, -270.3284710469133074 ) ) ;
#92966=CARTESIAN_POINT ( 'NONE',  ( 35.61928822639121961, -273.5201355730913519, -248.9481044826185610 ) ) ;
#92968=CARTESIAN_POINT ( 'NONE',  ( 32.03701970916272046, -280.7541136489308542, -247.2978729372258613 ) ) ;
#92969=CARTESIAN_POINT ( 'NONE',  ( -82.30077473322948833, -278.8558393342300405, -332.3828103828726626 ) ) ;
#92970=CARTESIAN_POINT ( 'NONE',  ( -99.70776026949154414, -274.4003459515403165, -231.4802998328978276 ) ) ;
#92971=CARTESIAN_POINT ( 'NONE',  ( -7.423735994318076514, -285.4935929101841339, -199.6099661249866983 ) ) ;
#92972=CARTESIAN_POINT ( 'NONE',  ( -110.7924322208123442, -292.1937882761323522, -279.4695738358672656 ) ) ;
#92973=CARTESIAN_POINT ( 'NONE',  ( -111.6675224746108910, -274.3645386415125813, -253.5649115234457440 ) ) ;
#92974=CARTESIAN_POINT ( 'NONE',  ( -27.07935770312077395, -275.4950453770099443, -194.4925801084156944 ) ) ;
#92976=CARTESIAN_POINT ( 'NONE',  ( 7.173461836765138600, -296.4447451395572557, -330.5790886482362794 ) ) ;
#92977=CARTESIAN_POINT ( 'NONE',  ( -101.9976272784508069, -282.0475739665027959, -308.0392218192928908 ) ) ;
#92978=CARTESIAN_POINT ( 'NONE',  ( -84.25010434077037758, -291.0938097002024847, -209.2583270212768980 ) ) ;
#92979=CARTESIAN_POINT ( 'NONE',  ( 14.66019250744243863, -272.8088843864364890, -216.8106748148640861 ) ) ;
#92980=CARTESIAN_POINT ( 'NONE',  ( -18.40079044007968179, -287.8922198484396517, -196.4981751354647770 ) ) ;
#92981=CARTESIAN_POINT ( 'NONE',  ( -70.34762781056551262, -290.5267630775066436, -204.9024683449930819 ) ) ;
#92982=ORIENTED_EDGE ( 'NONE', *, *, #61610, .T. ) ;
#92983=CARTESIAN_POINT ( 'NONE',  ( -105.9921682239077114, -288.6913632245349959, -304.0331896521166755 ) ) ;
#92984=CARTESIAN_POINT ( 'NONE',  ( -110.3582371856074502, -290.2080515255307205, -271.1813635585348266 ) ) ;
#92986=CARTESIAN_POINT ( 'NONE',  ( 22.74110137478180960, -287.9912237450164412, -222.6794168877924847 ) ) ;
#92987=CARTESIAN_POINT ( 'NONE',  ( -29.70699456949141037, -277.2862492517654687, -343.0329638910351377 ) ) ;
#92988=CARTESIAN_POINT ( 'NONE',  ( 17.33149365582932333, -293.2145233336383399, -324.2170639801052516 ) ) ;
#92989=CARTESIAN_POINT ( 'NONE',  ( -27.37707892590487901, -283.5802477009421523, -346.6641243589059513 ) ) ;
#92990=CARTESIAN_POINT ( 'NONE',  ( -80.92972839828624387, -285.8116507127966202, -206.8473613274224761 ) ) ;
#92991=CARTESIAN_POINT ( 'NONE',  ( -26.73551153524960000, -283.2469477231186374, -342.6592061572064836 ) ) ;
#92992=CARTESIAN_POINT ( 'NONE',  ( -13.02681774958086436, -91.53595701093347259, -360.0716045900807103 ) ) ;
#92993=CARTESIAN_POINT ( 'NONE',  ( -49.28614775429143435, -154.2781463013184862, -364.0998538831054816 ) ) ;
#92994=CARTESIAN_POINT ( 'NONE',  ( 201.3567858607021890, 292.7456558654927790, -53.99999999998547651 ) ) ;
#92995=CARTESIAN_POINT ( 'NONE',  ( 51.83402786492749215, -298.5460828057790081, -197.2694149549886049 ) ) ;
#92996=CARTESIAN_POINT ( 'NONE',  ( -43.49441721609006350, -272.8930728635862124, -197.2597297665910787 ) ) ;
#92997=CARTESIAN_POINT ( 'NONE',  ( -94.60996724338600927, -295.3619624269710471, -321.7604380975172944 ) ) ;
#92998=CARTESIAN_POINT ( 'NONE',  ( -75.80676782499371313, -208.7722911414634837, -353.9980045067355263 ) ) ;
#92999=CARTESIAN_POINT ( 'NONE',  ( -67.32683342920005032, -272.3518792780071749, -199.9751104633308216 ) ) ;
#93000=CARTESIAN_POINT ( 'NONE',  ( -102.3067754879293716, -298.8953373668895779, -234.4389178631257948 ) ) ;
#93001=CARTESIAN_POINT ( 'NONE',  ( 33.56211362645411356, -289.1233028498329531, -289.8864344532447035 ) ) ;
#93002=CARTESIAN_POINT ( 'NONE',  ( -108.0536675058858975, -291.8862691770031574, -251.0209074405942431 ) ) ;
#93004=CARTESIAN_POINT ( 'NONE',  ( -102.1242746498049883, -298.0348313538002003, -229.1781330127871854 ) ) ;
#93005=CARTESIAN_POINT ( 'NONE',  ( 35.02219564102053795, -288.1784640545204184, -280.5247508595293198 ) ) ;
#93006=CARTESIAN_POINT ( 'NONE',  ( 37.62863802467123264, -294.5667830215093090, -287.2611824451497569 ) ) ;
#93007=CARTESIAN_POINT ( 'NONE',  ( -1.990168916674266431, -295.0889824890612090, -338.6970246820822013 ) ) ;
#93008=CARTESIAN_POINT ( 'NONE',  ( 4.501905968599356989, -292.8007518216258518, -210.4818265202907241 ) ) ;
#93011=CARTESIAN_POINT ( 'NONE',  ( 32.85570986290937867, -277.8353555829073116, -298.4600837444673971 ) ) ;
#93013=CARTESIAN_POINT ( 'NONE',  ( -72.47311556739037997, -279.1074464091064442, -201.8971504870321212 ) ) ;
#93014=CARTESIAN_POINT ( 'NONE',  ( 28.24655160184914138, -276.9351408064773068, -303.0575238390532604 ) ) ;
#93015=CARTESIAN_POINT ( 'NONE',  ( -41.16451793200949538, -275.7649309509974387, -194.4190989342198463 ) ) ;
#93016=CARTESIAN_POINT ( 'NONE',  ( 2.607674430618251993, -274.5398401645783792, -334.3166156221017786 ) ) ;
#93017=CARTESIAN_POINT ( 'NONE',  ( -102.6270985249105792, -297.6506834490274400, -237.3590328285499425 ) ) ;
#93019=CARTESIAN_POINT ( 'NONE',  ( -110.7993925224842826, -295.1844250214292060, -265.9631248194395425 ) ) ;
#93021=CARTESIAN_POINT ( 'NONE',  ( -103.5496369594317798, -278.5323347258338345, -309.6578755844608963 ) ) ;
#93022=CARTESIAN_POINT ( 'NONE',  ( -9.986393335047198505, -276.8514442498514541, -338.0554580504505111 ) ) ;
#93024=CARTESIAN_POINT ( 'NONE',  ( 21.72021964146207651, -285.5794136726498778, -221.7299766454424059 ) ) ;
#93025=CARTESIAN_POINT ( 'NONE',  ( -112.1870949185858848, -274.6237131154039730, -264.8005701362116042 ) ) ;
#93026=CARTESIAN_POINT ( 'NONE',  ( 82.65242050738238788, -299.2778291467535610, -197.8518630440875086 ) ) ;
#93027=CARTESIAN_POINT ( 'NONE',  ( 32.82773924352123629, -286.4753734195056722, -249.6081724534010391 ) ) ;
#93029=CARTESIAN_POINT ( 'NONE',  ( -71.38812873509660051, -277.8360507084383926, -204.6291472771451083 ) ) ;
#93030=CARTESIAN_POINT ( 'NONE',  ( -106.0580368999380880, -277.4774390692523411, -243.8852364212453381 ) ) ;
#93031=CARTESIAN_POINT ( 'NONE',  ( -109.9380293223078127, -286.3097024978841318, -289.2464904731759248 ) ) ;
#93032=CARTESIAN_POINT ( 'NONE',  ( -18.90245113411350886, -278.0144995283549747, -341.4042358773270394 ) ) ;
#93034=CARTESIAN_POINT ( 'NONE',  ( -9.602886348971278352, -274.9345012027821440, -341.1038365056431303 ) ) ;
#93035=CARTESIAN_POINT ( 'NONE',  ( 15.51476457488577587, -275.4754439798660997, -219.7894674575021838 ) ) ;
#93036=CARTESIAN_POINT ( 'NONE',  ( 26.75531443692228706, -284.0789346990802073, -309.7230377057543933 ) ) ;
#93038=CARTESIAN_POINT ( 'NONE',  ( 26.24644227083116732, -290.0190225437839899, -311.2726156472203911 ) ) ;
#93039=CARTESIAN_POINT ( 'NONE',  ( -2.318195957178805777, -292.5889292846150056, -336.7378603377529203 ) ) ;
#93041=CARTESIAN_POINT ( 'NONE',  ( -51.64112410093822803, -272.5503579319287155, -198.2203552791679613 ) ) ;
#93042=CARTESIAN_POINT ( 'NONE',  ( 24.38120489545429592, -291.1285111381977231, -229.1161367624762590 ) ) ;
#93043=CARTESIAN_POINT ( 'NONE',  ( -78.59295187722810283, -208.2960365483323244, -357.4574221067172743 ) ) ;
#93045=CARTESIAN_POINT ( 'NONE',  ( -75.33541529648984181, -288.0290666810647622, -336.5365315481849962 ) ) ;
#93046=CARTESIAN_POINT ( 'NONE',  ( -104.8368268042791556, -285.7549519031385898, -300.2081997175055221 ) ) ;
#93047=CARTESIAN_POINT ( 'NONE',  ( -0.1917901401555877350, -284.7790798864511999, -204.0600822206697842 ) ) ;
#93049=CARTESIAN_POINT ( 'NONE',  ( -66.77873918761075345, -284.8708354357335679, -337.8198532561770548 ) ) ;
#93050=CARTESIAN_POINT ( 'NONE',  ( -37.53069501245036577, -283.8574474257169982, -343.5348076018982511 ) ) ;
#93051=CARTESIAN_POINT ( 'NONE',  ( -93.50266628165103100, -293.2283898004811249, -220.1181813164247671 ) ) ;
#93052=CARTESIAN_POINT ( 'NONE',  ( 29.97862184496998950, -273.1817012103730917, -236.0494808218185199 ) ) ;
#93053=CARTESIAN_POINT ( 'NONE',  ( -46.88258587029088886, -274.2674179150606051, -193.9758066280504352 ) ) ;
#93054=CARTESIAN_POINT ( 'NONE',  ( -110.2370002989357829, -288.8864269982775568, -250.4226518658473424 ) ) ;
#93055=CARTESIAN_POINT ( 'NONE',  ( -17.35789933755228986, -276.8011508202511095, -344.7227190005884268 ) ) ;
#93056=CARTESIAN_POINT ( 'NONE',  ( -25.93166203061819886, -296.8860210818939436, -344.1287113486369549 ) ) ;
#93059=CARTESIAN_POINT ( 'NONE',  ( -107.8698714033939865, -282.9648861105554261, -291.0705614155507988 ) ) ;
#93060=CARTESIAN_POINT ( 'NONE',  ( -76.42789811154166557, -277.5296757881509393, -206.2910869157447848 ) ) ;
#93062=CARTESIAN_POINT ( 'NONE',  ( -108.5128642368318452, -271.3854633129844274, -242.6953564316367249 ) ) ;
#93063=CARTESIAN_POINT ( 'NONE',  ( -97.73771417988540122, -277.3285540484964713, -311.5462385349812848 ) ) ;
#93064=CARTESIAN_POINT ( 'NONE',  ( -28.03782170694745446, -293.6923771513891097, -197.2062251197209832 ) ) ;
#93065=CARTESIAN_POINT ( 'NONE',  ( -19.81345734441296003, -279.1925818874099718, -195.6456432837802026 ) ) ;
#93066=CARTESIAN_POINT ( 'NONE',  ( 21.98831031567865324, -293.8944293638078875, -227.4054485807543529 ) ) ;
#93068=CARTESIAN_POINT ( 'NONE',  ( -47.54909627123434035, -296.4944988658038483, -346.1839861415475639 ) ) ;
#93069=CARTESIAN_POINT ( 'NONE',  ( -99.89569917015704448, -296.9044136526502484, -232.6330814757076553 ) ) ;
#93070=CARTESIAN_POINT ( 'NONE',  ( -79.27202385440597254, -291.6177795216910908, -332.6076168281423406 ) ) ;
#93071=CARTESIAN_POINT ( 'NONE',  ( -106.6800326892034576, -285.1484475823513662, -236.8768583651322501 ) ) ;
#93072=CARTESIAN_POINT ( 'NONE',  ( -78.15589703447028569, -271.6491471499148247, -206.5292543873677857 ) ) ;
#93073=CARTESIAN_POINT ( 'NONE',  ( 39.34725525326049933, -287.4719423508337854, -277.2751708469426148 ) ) ;
#93074=CARTESIAN_POINT ( 'NONE',  ( -84.49587380032733108, -281.3795587611379005, -212.4294362897949497 ) ) ;
#93075=CARTESIAN_POINT ( 'NONE',  ( -44.03398219609740494, -285.0242068742987840, -197.4322361261056358 ) ) ;
#93076=CARTESIAN_POINT ( 'NONE',  ( -12.90021255846555803, -286.7344887951414876, -341.3212026923465032 ) ) ;
#93077=CARTESIAN_POINT ( 'NONE',  ( 65.71450562203199297, 45.78484130816451625, -315.1169351998001389 ) ) ;
#93078=CARTESIAN_POINT ( 'NONE',  ( -35.92599322437101250, -285.5780356783108118, -197.3132965515756041 ) ) ;
#93079=CARTESIAN_POINT ( 'NONE',  ( -1.732611843408993213, -283.5332029453692826, -338.3670959927394506 ) ) ;
#93080=CARTESIAN_POINT ( 'NONE',  ( -92.63425842660852538, -290.3428300924794598, -217.0355948503207628 ) ) ;
#93081=CARTESIAN_POINT ( 'NONE',  ( -110.5741047771483068, -280.4190676228725465, -249.3027389963448854 ) ) ;
#93082=CARTESIAN_POINT ( 'NONE',  ( -68.48720090725359455, -280.9666015271668584, -200.4665246857018701 ) ) ;
#93083=CARTESIAN_POINT ( 'NONE',  ( 33.45610174191814679, -281.1500165434163137, -252.5150661209417535 ) ) ;
#93084=CARTESIAN_POINT ( 'NONE',  ( 35.85051572032931944, -277.7632188498862433, -286.7872602501676056 ) ) ;
#93085=CARTESIAN_POINT ( 'NONE',  ( -1.967479606768923972, -294.5967149062826707, -338.7545717812208750 ) ) ;
#93086=CARTESIAN_POINT ( 'NONE',  ( 21.64198774099219946, -286.2026102814044179, -316.1286215399728690 ) ) ;
#93088=CARTESIAN_POINT ( 'NONE',  ( -95.06833701218657495, -292.8311306700215368, -220.6010848072217243 ) ) ;
#93089=CARTESIAN_POINT ( 'NONE',  ( -94.68454819221240371, -296.1147713699570545, -224.6881078929420426 ) ) ;
#93091=CARTESIAN_POINT ( 'NONE',  ( -38.89100651573278355, -284.9918561178558321, -344.7977351325462223 ) ) ;
#93092=CARTESIAN_POINT ( 'NONE',  ( -93.96163396402897661, -295.5661548307197677, -316.4922725720511494 ) ) ;
#93093=CARTESIAN_POINT ( 'NONE',  ( 21.06605969209302742, -293.9588272986272273, -220.6417030200217653 ) ) ;
#93094=CARTESIAN_POINT ( 'NONE',  ( -90.81036690005215917, -284.4876784674281112, -320.2108355532662358 ) ) ;
#93095=CARTESIAN_POINT ( 'NONE',  ( 24.29811901751222791, -274.0007147202811097, -224.6079442208886974 ) ) ;
#93096=CARTESIAN_POINT ( 'NONE',  ( -59.98933079607509455, -289.9895726250152848, -343.8485156196079515 ) ) ;
#93097=CARTESIAN_POINT ( 'NONE',  ( -83.15545261262880672, -281.8111243733034144, -330.7710974910717709 ) ) ;
#93098=CARTESIAN_POINT ( 'NONE',  ( 26.38375981320465868, -287.3966455321070157, -234.6044379002715061 ) ) ;
#93101=CARTESIAN_POINT ( 'NONE',  ( 5.919522898407217681, -59.40102248639579585, -350.9217243335569378 ) ) ;
#93102=CARTESIAN_POINT ( 'NONE',  ( -69.85430415644619018, -271.1237833571632905, -202.7746430608542312 ) ) ;
#93103=CARTESIAN_POINT ( 'NONE',  ( -66.12383106651755327, -278.8627301550951074, -203.0853455465862965 ) ) ;
#93105=CARTESIAN_POINT ( 'NONE',  ( -1.804242960465771040, -279.4551587318641737, -206.2415795241771264 ) ) ;
#93106=CARTESIAN_POINT ( 'NONE',  ( 38.90381832115386374, -275.0862650558409541, -259.7608723289450268 ) ) ;
#93107=CARTESIAN_POINT ( 'NONE',  ( 200.8605831797993062, 286.2175693065611313, -96.73721376744219924 ) ) ;
#93108=CARTESIAN_POINT ( 'NONE',  ( -25.46910903888736044, -278.7753607374153830, -194.8783525826691516 ) ) ;
#93109=CARTESIAN_POINT ( 'NONE',  ( 6.539107288121340567, -280.4725110617044948, -330.7458970281825259 ) ) ;
#93110=CARTESIAN_POINT ( 'NONE',  ( -87.91408334400087199, -297.5075524510115770, -327.1450434393960904 ) ) ;
#93111=CARTESIAN_POINT ( 'NONE',  ( 10.33641514772100400, -294.8652731128516393, -325.7216252528195923 ) ) ;
#93113=CARTESIAN_POINT ( 'NONE',  ( -91.10862421313703408, -289.9527849138713691, -220.2390095541911990 ) ) ;
#93114=CARTESIAN_POINT ( 'NONE',  ( 23.54704104386278374, -275.5756721324939917, -223.3729548992785965 ) ) ;
#93115=CARTESIAN_POINT ( 'NONE',  ( -74.27338320858079612, -273.5467846817364261, -207.3339124957474837 ) ) ;
#93119=CARTESIAN_POINT ( 'NONE',  ( 9.463374133154447421, -281.7927296435440212, -213.8723435883612467 ) ) ;
#93120=CARTESIAN_POINT ( 'NONE',  ( -11.87042734609747008, -282.1392417980473510, -198.7154593833747356 ) ) ;
#93121=CARTESIAN_POINT ( 'NONE',  ( -97.73315469419704016, -283.0350247642923591, -311.8775397146829960 ) ) ;
#93122=CARTESIAN_POINT ( 'NONE',  ( 32.21957138567422874, -283.0708036584871365, -244.2889745518489519 ) ) ;
#93123=CARTESIAN_POINT ( 'NONE',  ( 35.71033753081844253, -273.9052576440688540, -260.6602135802889393 ) ) ;
#93126=CARTESIAN_POINT ( 'NONE',  ( -42.78450690990434424, -277.9220227374310070, -347.0066310598303403 ) ) ;
#93130=CARTESIAN_POINT ( 'NONE',  ( -111.9668163267544685, -286.3936198589705100, -281.1929735122029115 ) ) ;
#93131=CARTESIAN_POINT ( 'NONE',  ( 30.00838957883324198, -292.3649631812576217, -241.6558253157915885 ) ) ;
#93132=CARTESIAN_POINT ( 'NONE',  ( -36.09682285605904895, -288.3855521207364063, -347.2622014783534041 ) ) ;
#93133=ADVANCED_FACE ( 'NONE', ( #56683 ), #55175, .F. ) ;
#93134=CARTESIAN_POINT ( 'NONE',  ( -109.0042749793001065, -283.0329551182600198, -251.8557300806889998 ) ) ;
#93135=CARTESIAN_POINT ( 'NONE',  ( -94.56889780037019477, -283.7761620456114429, -224.0764497911150954 ) ) ;
#93136=CARTESIAN_POINT ( 'NONE',  ( -40.01690294164932027, -287.3259529322153298, -344.3763600051889853 ) ) ;
#93137=CARTESIAN_POINT ( 'NONE',  ( 8.051511651281192172, -283.6210873779231179, -328.1026085126521821 ) ) ;
#93138=CARTESIAN_POINT ( 'NONE',  ( 0.2165205984923093130, -272.5520562238553453, -205.4279655805774780 ) ) ;
#93139=CARTESIAN_POINT ( 'NONE',  ( -103.3372930389460862, -283.4536427480870771, -232.1639501995029491 ) ) ;
#93140=CARTESIAN_POINT ( 'NONE',  ( -66.13250785542608412, -297.4290927360626711, -339.6287572299213480 ) ) ;
#93141=CARTESIAN_POINT ( 'NONE',  ( -109.9436069472899078, -282.8039599072970418, -250.6980402026196089 ) ) ;
#93142=CARTESIAN_POINT ( 'NONE',  ( -94.98345866781528457, -280.1284964571382829, -225.1653147560482751 ) ) ;
#93143=CARTESIAN_POINT ( 'NONE',  ( 28.51277332754802885, -289.0702739978530076, -234.0148528554576615 ) ) ;
#93146=CARTESIAN_POINT ( 'NONE',  ( 34.08324848750269354, -295.1537932293272206, -245.5494747685061441 ) ) ;
#93148=CARTESIAN_POINT ( 'NONE',  ( -46.16807715613111185, -275.1638176601100554, -344.8919588464014510 ) ) ;
#93149=CARTESIAN_POINT ( 'NONE',  ( -101.5434026802915497, -290.3065588331792810, -228.0483588684395500 ) ) ;
#93150=CARTESIAN_POINT ( 'NONE',  ( -2.787021886263308712, -292.9871755478962996, -335.5716587581698604 ) ) ;
#93151=CARTESIAN_POINT ( 'NONE',  ( -85.79684564789548062, -278.0491499384419285, -215.1040609725515651 ) ) ;
#93152=CARTESIAN_POINT ( 'NONE',  ( -111.7817001273664914, -270.6323071128609854, -270.3367258320721476 ) ) ;
#93153=CARTESIAN_POINT ( 'NONE',  ( -82.04217990329473764, -292.7436585343715478, -211.9605230838566854 ) ) ;
#93154=CARTESIAN_POINT ( 'NONE',  ( 10.59707575819634329, -277.1948066931274184, -210.1954327657594490 ) ) ;
#93155=CARTESIAN_POINT ( 'NONE',  ( -1.053108605244923890, -293.0594187530589920, -337.5014653714754900 ) ) ;
#93156=CARTESIAN_POINT ( 'NONE',  ( 23.42002051306367250, -289.7295423746724055, -312.2696011030996601 ) ) ;
#93157=CARTESIAN_POINT ( 'NONE',  ( -7.566342243576914761, -290.6769990101252574, -200.4370257377942153 ) ) ;
#93159=CARTESIAN_POINT ( 'NONE',  ( -45.40916316825265397, -290.5816462755353768, -343.5068010866767167 ) ) ;
#93162=CARTESIAN_POINT ( 'NONE',  ( -13.22502340328375325, -289.5335340590501687, -339.4334542002155217 ) ) ;
#93164=CARTESIAN_POINT ( 'NONE',  ( 144.7857639756989272, -299.5541904835127980, -195.3611179825600175 ) ) ;
#93165=CARTESIAN_POINT ( 'NONE',  ( -106.1500589670266663, -291.3212879949576291, -304.1479227005356734 ) ) ;
#93166=CARTESIAN_POINT ( 'NONE',  ( 24.93581247954994851, -278.9994757435598558, -227.8445861780787425 ) ) ;
#93167=CARTESIAN_POINT ( 'NONE',  ( -102.4095665108567346, -291.0029521426351948, -237.1558258851979417 ) ) ;
#93168=CARTESIAN_POINT ( 'NONE',  ( -28.23171886346071346, -280.4978958992466005, -193.8696082705689889 ) ) ;
#93169=CARTESIAN_POINT ( 'NONE',  ( 36.45719177757317198, -281.4957414389079418, -292.4412136093652066 ) ) ;
#93170=CARTESIAN_POINT ( 'NONE',  ( 28.78206567304079400, -286.0228955512463926, -305.8643518758161690 ) ) ;
#93172=CARTESIAN_POINT ( 'NONE',  ( 21.13964999677434164, -280.3255648648585066, -316.0863535890235312 ) ) ;
#93173=CARTESIAN_POINT ( 'NONE',  ( -110.4054452489891389, -282.7694014932187656, -253.4292013009956008 ) ) ;
#93174=DIRECTION ( 'NONE',  ( -1.000000000000000000, -0.000000000000000000, -0.000000000000000000 ) ) ;
#93175=CARTESIAN_POINT ( 'NONE',  ( -6.492755947594490706, -278.9298411078752906, -200.5540615095610519 ) ) ;
#93176=CARTESIAN_POINT ( 'NONE',  ( 23.62410741522981539, -285.8494631136304633, -223.8136448187762824 ) ) ;
#93177=CARTESIAN_POINT ( 'NONE',  ( 19.11695759141926487, -275.6969973515500101, -223.8313243444474097 ) ) ;
#93179=CARTESIAN_POINT ( 'NONE',  ( -37.57268920814497193, -293.6493788064684054, -196.5488969111771951 ) ) ;
#93180=CARTESIAN_POINT ( 'NONE',  ( 19.58466405522391085, -276.2800653926019550, -219.3128497882555052 ) ) ;
#93181=CARTESIAN_POINT ( 'NONE',  ( -83.02329073002005089, -277.3637853461275427, -327.3935549608236215 ) ) ;
#93182=CARTESIAN_POINT ( 'NONE',  ( -104.6110077779511158, -291.2045613214863806, -232.8932617215579626 ) ) ;
#93183=CARTESIAN_POINT ( 'NONE',  ( 33.97680217068388941, -279.3094003535211982, -245.2450221761572209 ) ) ;
#93184=CARTESIAN_POINT ( 'NONE',  ( -86.51140065456102946, -291.2244386477576086, -211.0353227272537993 ) ) ;
#93185=CARTESIAN_POINT ( 'NONE',  ( -77.37378323696128746, -290.5592624433946867, -209.0354237774879209 ) ) ;
#93186=CARTESIAN_POINT ( 'NONE',  ( -50.15165102018294618, -293.2153406318451516, -344.3116058711942173 ) ) ;
#93189=CARTESIAN_POINT ( 'NONE',  ( -41.59015181807210126, -291.5049936054648470, -197.3733166614469212 ) ) ;
#93191=CARTESIAN_POINT ( 'NONE',  ( 17.40634833298269157, -272.4094976428775681, -226.7417163044926838 ) ) ;
#93192=CARTESIAN_POINT ( 'NONE',  ( -108.6655231179850318, -295.9736987428496491, -241.8329011001955564 ) ) ;
#93193=CARTESIAN_POINT ( 'NONE',  ( -111.8830607454059702, -286.0841991713620587, -253.1308007344528903 ) ) ;
#93194=CARTESIAN_POINT ( 'NONE',  ( 28.81085032344271113, -286.9686574778456247, -239.4930102783042685 ) ) ;
#93195=CARTESIAN_POINT ( 'NONE',  ( 31.76181859306231914, -276.7340999501711849, -244.7601130837306300 ) ) ;
#93196=CARTESIAN_POINT ( 'NONE',  ( 32.10680081907952399, -291.9317833439520200, -297.8657594590737290 ) ) ;
#93197=CARTESIAN_POINT ( 'NONE',  ( -104.8518433362911395, -297.9077449048450603, -300.8236596657920927 ) ) ;
#93198=CARTESIAN_POINT ( 'NONE',  ( -11.12647552631010583, -275.4976091959406403, -338.9168799870798807 ) ) ;
#93199=VERTEX_POINT ( 'NONE', #20677 ) ;
#93201=CARTESIAN_POINT ( 'NONE',  ( -70.80251967740142049, -295.1481565284537965, -339.7017943972039120 ) ) ;
#93202=CARTESIAN_POINT ( 'NONE',  ( 24.72336272961265990, -290.0318261111931974, -311.4848030009810600 ) ) ;
#93203=CARTESIAN_POINT ( 'NONE',  ( -39.82724512258611327, -296.0207706036652553, -195.3991614904663834 ) ) ;
#93204=CARTESIAN_POINT ( 'NONE',  ( 10.18782403219246291, -289.0279254370976787, -325.9693646830477292 ) ) ;
#93206=CARTESIAN_POINT ( 'NONE',  ( -42.40253659557587440, -279.0485423625825661, -193.7634147053533979 ) ) ;
#93207=CARTESIAN_POINT ( 'NONE',  ( -72.02063264983242163, -296.1500618565520995, -338.9955439375869446 ) ) ;
#93208=CARTESIAN_POINT ( 'NONE',  ( -94.54158972101012637, -288.0092790155520106, -320.0448991685104829 ) ) ;
#93209=CARTESIAN_POINT ( 'NONE',  ( -97.38827637270021853, -296.2396469624651445, -318.5499442493396032 ) ) ;
#93210=CARTESIAN_POINT ( 'NONE',  ( 32.77166751017819735, -294.1557543438928519, -290.8071271024535349 ) ) ;
#93214=CARTESIAN_POINT ( 'NONE',  ( 23.29855873569807301, -288.4488359496038470, -224.0205176423681621 ) ) ;
#93215=CARTESIAN_POINT ( 'NONE',  ( 108.6256185021308909, -297.2649936051623740, -190.4191791630918544 ) ) ;
#93216=CARTESIAN_POINT ( 'NONE',  ( -99.34076080730291380, -278.5059570782535161, -224.8479177433979146 ) ) ;
#93217=CARTESIAN_POINT ( 'NONE',  ( -90.17095008656997379, -285.8008580657005950, -323.4347564590783577 ) ) ;
#93218=CARTESIAN_POINT ( 'NONE',  ( -40.77171308501063862, -284.5846698096116825, -193.9755741433193066 ) ) ;
#93219=CARTESIAN_POINT ( 'NONE',  ( 36.88578273420901610, -285.7130431712475342, -276.6264036958883707 ) ) ;
#93220=CARTESIAN_POINT ( 'NONE',  ( 33.04566781476661674, -277.7756270724763681, -298.5370105251740256 ) ) ;
#93222=CARTESIAN_POINT ( 'NONE',  ( -87.09553140190301690, -277.7687916458238533, -323.7798064125101973 ) ) ;
#93223=CARTESIAN_POINT ( 'NONE',  ( -87.59468463720851616, -278.6769310511675144, -217.2013385646314418 ) ) ;
#93224=CARTESIAN_POINT ( 'NONE',  ( -31.29819022591435385, -275.2064340972066248, -193.8954962995532014 ) ) ;
#93225=CARTESIAN_POINT ( 'NONE',  ( -112.6031698240258407, -277.5273917225454170, -256.0179914359422355 ) ) ;
#93226=CARTESIAN_POINT ( 'NONE',  ( 191.7767904288494378, 277.8504399066188739, -124.6329446178930596 ) ) ;
#93227=CARTESIAN_POINT ( 'NONE',  ( -95.85613748882796870, -274.1654335761859898, -220.6530411189235963 ) ) ;
#93229=CARTESIAN_POINT ( 'NONE',  ( -34.09648980177933453, -299.5172960264183644, -193.9495737372290876 ) ) ;
#93230=CARTESIAN_POINT ( 'NONE',  ( -110.4683760289727132, -281.2662352645559167, -253.7030783399848985 ) ) ;
#93233=CARTESIAN_POINT ( 'NONE',  ( -77.22873350587327934, -286.5835819542757577, -208.7927466873358355 ) ) ;
#93234=CARTESIAN_POINT ( 'NONE',  ( -103.1738990033099412, -286.8133712669272768, -232.3078380909712166 ) ) ;
#93235=CARTESIAN_POINT ( 'NONE',  ( 5.898248701612346601, -287.7971725074971232, -329.3665380403085123 ) ) ;
#93236=CARTESIAN_POINT ( 'NONE',  ( -102.8689525709657033, -283.5324068435402296, -310.6811637466795446 ) ) ;
#93237=CARTESIAN_POINT ( 'NONE',  ( -65.09831104353023079, -278.0831800794574633, -201.9797538079899653 ) ) ;
#93238=CARTESIAN_POINT ( 'NONE',  ( 22.98168641837745696, -288.8168386370695089, -227.0083982521929613 ) ) ;
#93239=CARTESIAN_POINT ( 'NONE',  ( 27.45557632168236495, -280.5064568608930244, -305.4612706237875273 ) ) ;
#93240=CARTESIAN_POINT ( 'NONE',  ( -61.93920510712349170, -278.6937564520988531, -339.6698644878733830 ) ) ;
#93241=CARTESIAN_POINT ( 'NONE',  ( 31.32174707990530749, -276.3786278270961816, -295.4745358232566446 ) ) ;
#93242=CARTESIAN_POINT ( 'NONE',  ( -74.24954294168227875, -288.3264413884608643, -337.5014992780453440 ) ) ;
#93243=CARTESIAN_POINT ( 'NONE',  ( 2.020217356878742265, -283.3420920574939714, -336.3520133569123800 ) ) ;
#93244=CARTESIAN_POINT ( 'NONE',  ( -111.8138159825695226, -284.8018507506114361, -289.7376920111759091 ) ) ;
#93245=CARTESIAN_POINT ( 'NONE',  ( 2.702210927790849926, -280.7721714879038473, -209.2637113911700055 ) ) ;
#93249=CARTESIAN_POINT ( 'NONE',  ( -34.68600440572502919, -290.8795236966608400, -346.0793638883434937 ) ) ;
#93250=CARTESIAN_POINT ( 'NONE',  ( -104.7295647735549835, -288.7656358596715904, -306.5850599277380297 ) ) ;
#93251=CARTESIAN_POINT ( 'NONE',  ( -110.5765481139782196, -271.6469838737972964, -267.6165227046483892 ) ) ;
#93252=CARTESIAN_POINT ( 'NONE',  ( -8.434063738488317696, -294.0322482892400444, -341.6752324797988081 ) ) ;
#93253=CARTESIAN_POINT ( 'NONE',  ( -80.83214107322541508, -288.1339781007159786, -329.9165559745742939 ) ) ;
#93254=CARTESIAN_POINT ( 'NONE',  ( 36.54783670435628551, -291.7257453472619204, -265.2686451037963593 ) ) ;
#93255=CARTESIAN_POINT ( 'NONE',  ( 10.38504338120647752, -289.5814988634830343, -326.1893255028828662 ) ) ;
#93256=CARTESIAN_POINT ( 'NONE',  ( -95.99890600148557951, -287.6948066931273615, -223.6242672951989618 ) ) ;
#93257=CARTESIAN_POINT ( 'NONE',  ( -5.167333334178064064, -290.6288725286586327, -338.1233663568738734 ) ) ;
#93258=CARTESIAN_POINT ( 'NONE',  ( -47.47051817817688146, -289.9236734089861898, -195.8274979675384770 ) ) ;
#93259=CARTESIAN_POINT ( 'NONE',  ( -91.72135787159771780, -293.2776441320560252, -218.6364017236690813 ) ) ;
#93260=CARTESIAN_POINT ( 'NONE',  ( -89.05196576053039337, -284.7421202252446619, -322.2922591787229294 ) ) ;
#93261=CARTESIAN_POINT ( 'NONE',  ( 3.132385292289554979, -294.5941410494969546, -206.9600567826655322 ) ) ;
#93264=CARTESIAN_POINT ( 'NONE',  ( -80.33314189798755933, -275.4532652014053156, -208.4097262069114151 ) ) ;
#93265=CARTESIAN_POINT ( 'NONE',  ( 10.00543177577010923, -281.5774892429994907, -326.2027343632244651 ) ) ;
#93266=CARTESIAN_POINT ( 'NONE',  ( -109.6971933644954476, -282.2975897089835371, -290.1500638363548319 ) ) ;
#93267=CARTESIAN_POINT ( 'NONE',  ( -72.01034808124663300, -294.6960513229583967, -338.9340256811822769 ) ) ;
#93268=CARTESIAN_POINT ( 'NONE',  ( -31.23405102780345644, -272.3701744045952182, -196.5873909089060589 ) ) ;
#93269=CARTESIAN_POINT ( 'NONE',  ( -72.35265904695719996, -275.5989812871129629, -336.0683205116607724 ) ) ;
#93270=CARTESIAN_POINT ( 'NONE',  ( -108.4424471954553297, -297.6228236523456303, -289.0099496874532861 ) ) ;
#93271=CARTESIAN_POINT ( 'NONE',  ( -69.86435409441874356, -272.2070019753833776, -201.2028845899655209 ) ) ;
#93272=CARTESIAN_POINT ( 'NONE',  ( -55.93479655009908669, -296.7214404505634775, -341.6155472440119070 ) ) ;
#93274=CARTESIAN_POINT ( 'NONE',  ( -68.12476745079561624, -298.4401372515159210, -203.9772147238924731 ) ) ;
#93276=CARTESIAN_POINT ( 'NONE',  ( 4.292381753523367038, -284.6301468204551952, -207.4896404317160545 ) ) ;
#93277=CARTESIAN_POINT ( 'NONE',  ( -52.63508903548208906, -297.8508622236386145, -198.9291775584406423 ) ) ;
#93278=CARTESIAN_POINT ( 'NONE',  ( -33.72732828725057175, -286.0964577531777309, -193.4459938768536915 ) ) ;
#93279=CARTESIAN_POINT ( 'NONE',  ( 37.48286012622866537, -287.4457620360851138, -288.5007465700223861 ) ) ;
#93280=CARTESIAN_POINT ( 'NONE',  ( 14.36870489703889930, -296.3092717248750319, -325.1738976320864936 ) ) ;
#93281=CARTESIAN_POINT ( 'NONE',  ( -6.491756904026782848, -290.4580877301786472, -202.1826064635637579 ) ) ;
#93282=CARTESIAN_POINT ( 'NONE',  ( -31.07670702468217883, -279.3264374759253315, -193.7258460152913813 ) ) ;
#93283=CARTESIAN_POINT ( 'NONE',  ( -20.25526795762938548, -292.3380690714490129, -345.3683826091709648 ) ) ;
#93285=CARTESIAN_POINT ( 'NONE',  ( -17.04743965292329477, -285.1148594994880909, -199.7723608643943578 ) ) ;
#93288=CARTESIAN_POINT ( 'NONE',  ( 13.49318756761085858, -286.3408371416484215, -325.5752490717426326 ) ) ;
#93289=CARTESIAN_POINT ( 'NONE',  ( -63.38060158658408483, -299.3074077254074155, -201.2533270183511149 ) ) ;
#93290=CARTESIAN_POINT ( 'NONE',  ( -81.91000493751778322, -280.8831249738808538, -208.2944401444763969 ) ) ;
#93291=CARTESIAN_POINT ( 'NONE',  ( -107.3509338238933708, -294.9352257619309512, -242.3442498308210418 ) ) ;
#93292=CARTESIAN_POINT ( 'NONE',  ( 21.81193784710044525, -282.1508164467197730, -313.1592329575821623 ) ) ;
#93293=CARTESIAN_POINT ( 'NONE',  ( -95.58010622918196475, -296.0383599629009268, -320.7326184498346606 ) ) ;
#93294=CARTESIAN_POINT ( 'NONE',  ( 52.71383863060632535, -300.7196638740886101, -196.6439986017678336 ) ) ;
#93295=CARTESIAN_POINT ( 'NONE',  ( 36.61912566161930727, -285.4341290740508157, -254.8351783483052202 ) ) ;
#93297=CARTESIAN_POINT ( 'NONE',  ( 34.67203289475921935, -283.2820090330147309, -249.3622583848950285 ) ) ;
#93298=CARTESIAN_POINT ( 'NONE',  ( -109.1177205576019986, -295.4187948998850857, -284.9704867222752682 ) ) ;
#93300=FACE_OUTER_BOUND ( 'NONE', #56442, .T. ) ;
#93301=CARTESIAN_POINT ( 'NONE',  ( -2.839196279003161738, -284.5737230785408656, -336.5677667542994413 ) ) ;
#93303=CARTESIAN_POINT ( 'NONE',  ( -110.4683760289727132, -293.8380690714490129, -287.0191576251351080 ) ) ;
#93304=CARTESIAN_POINT ( 'NONE',  ( 39.46971532985821085, -274.7237430993175167, -268.3202173590611324 ) ) ;
#93305=CARTESIAN_POINT ( 'NONE',  ( 34.21691060942654872, -293.1950517655050135, -255.9262562289091250 ) ) ;
#93306=CARTESIAN_POINT ( 'NONE',  ( 35.01130376753191342, -282.8885804716250618, -256.3036385444580674 ) ) ;
#93307=CARTESIAN_POINT ( 'NONE',  ( 34.28070615558948475, -276.9199999627544457, -252.5658563827510363 ) ) ;
#93308=CARTESIAN_POINT ( 'NONE',  ( 22.78437203438852521, -283.7843979327710713, -317.1934895650267094 ) ) ;
#93309=CARTESIAN_POINT ( 'NONE',  ( 33.84443509571659092, -280.1117888279570707, -252.4308431735550187 ) ) ;
#93310=CARTESIAN_POINT ( 'NONE',  ( -111.6057779990163255, -280.6915240885984417, -259.5190959958131884 ) ) ;
#93311=CARTESIAN_POINT ( 'NONE',  ( -35.47191091186855516, -298.0749566773375250, -193.3611179589730114 ) ) ;
#93312=CARTESIAN_POINT ( 'NONE',  ( 39.63091839200972544, -275.3597932469244824, -268.3078272955459624 ) ) ;
#93313=CARTESIAN_POINT ( 'NONE',  ( 36.26555900383650055, -295.6202948441273293, -281.8005251867387528 ) ) ;
#93316=CARTESIAN_POINT ( 'NONE',  ( 37.38402868702716120, -291.8516765407208027, -282.9444184885438744 ) ) ;
#93317=CARTESIAN_POINT ( 'NONE',  ( -85.34588000748786385, -272.8754448530427794, -215.2156834523604516 ) ) ;
#93318=CARTESIAN_POINT ( 'NONE',  ( 36.79108678526437615, -295.3011602620046006, -288.5000327931616084 ) ) ;
#93319=CARTESIAN_POINT ( 'NONE',  ( -44.87335835601073342, -293.1640258718359746, -194.0766977850057060 ) ) ;
#93320=CARTESIAN_POINT ( 'NONE',  ( -74.43204382939174479, -291.5467401000939844, -335.3707720548350721 ) ) ;
#93321=CARTESIAN_POINT ( 'NONE',  ( -110.6789582931641576, -276.7444154536066776, -255.4081223257527142 ) ) ;
#93322=CARTESIAN_POINT ( 'NONE',  ( -8.151917034199209766, -278.5870405011910975, -338.8531802630988636 ) ) ;
#93323=CARTESIAN_POINT ( 'NONE',  ( -23.27013289461709533, -292.9508071713839854, -343.5116525890737194 ) ) ;
#93324=CARTESIAN_POINT ( 'NONE',  ( 29.61888168925902320, -282.9460514792619392, -234.8009771056352690 ) ) ;
#93325=CARTESIAN_POINT ( 'NONE',  ( -57.46609736118185907, -284.7066698001199256, -199.8154861949709868 ) ) ;
#93326=CARTESIAN_POINT ( 'NONE',  ( 27.36018454229470720, -24.35185690934844516, -343.9753583313619174 ) ) ;
#93328=CARTESIAN_POINT ( 'NONE',  ( -78.39201907150409454, -283.2884260675377845, -330.7511734665007452 ) ) ;
#93329=CARTESIAN_POINT ( 'NONE',  ( -68.55933889872609655, -280.7311369922315407, -200.2971523889772243 ) ) ;
#93330=CARTESIAN_POINT ( 'NONE',  ( -111.4944852100812227, -283.1047022657428442, -289.6322467330157338 ) ) ;
#93331=CARTESIAN_POINT ( 'NONE',  ( -53.72199561105000498, -280.7882851932529888, -195.3100066458064248 ) ) ;
#93333=CARTESIAN_POINT ( 'NONE',  ( -45.55556898334211979, -278.6744293241106902, -346.2769971086904093 ) ) ;
#93334=CARTESIAN_POINT ( 'NONE',  ( 34.45848030099739390, -296.0519495502701943, -270.3284710469131937 ) ) ;
#93337=CARTESIAN_POINT ( 'NONE',  ( -97.77667142547001333, -275.1561204509398522, -226.1428834626578066 ) ) ;
#93338=CARTESIAN_POINT ( 'NONE',  ( -35.59969422421068685, -278.0941927101180795, -195.7239614331422786 ) ) ;
#93339=CARTESIAN_POINT ( 'NONE',  ( -111.8696634739424098, -292.1236695618717931, -285.2444201393055891 ) ) ;
#93340=CARTESIAN_POINT ( 'NONE',  ( 12.41819523943533632, -293.6858028803654292, -323.9827584333213508 ) ) ;
#93341=CARTESIAN_POINT ( 'NONE',  ( -38.92519833999234891, -288.5791756989824535, -347.2832827784969822 ) ) ;
#93343=CARTESIAN_POINT ( 'NONE',  ( 29.05361676038690177, -292.6230298726919159, -308.2868464497824448 ) ) ;
#93344=CARTESIAN_POINT ( 'NONE',  ( -49.53384484530918286, -284.2941206061042863, -197.5231245158441311 ) ) ;
#93345=CARTESIAN_POINT ( 'NONE',  ( -41.68845706475383395, -293.8573768313712549, -196.2025939599754736 ) ) ;
#93346=CARTESIAN_POINT ( 'NONE',  ( 18.31239808476545150, -285.3499201719639018, -222.0565725876165288 ) ) ;
#93347=CARTESIAN_POINT ( 'NONE',  ( 24.55476209715605052, -283.4128955366576292, -310.0788312290978865 ) ) ;
#93348=CARTESIAN_POINT ( 'NONE',  ( -113.4345562563489551, -291.6254167333763689, -259.8375318194370607 ) ) ;
#93349=CARTESIAN_POINT ( 'NONE',  ( 19.72015016035604873, -281.4004084286986540, -224.7329064950718305 ) ) ;
#93350=CARTESIAN_POINT ( 'NONE',  ( 36.70877110848037717, -292.5938523750085665, -289.9707184176549504 ) ) ;
#93351=CARTESIAN_POINT ( 'NONE',  ( 37.95210925836853733, -288.5471032869760393, -285.6908632237289680 ) ) ;
#93352=CARTESIAN_POINT ( 'NONE',  ( -28.97763250525009227, -289.4413137809881960, -346.8970783663022530 ) ) ;
#93353=CARTESIAN_POINT ( 'NONE',  ( -4.596464110547775483, -286.6627916813097272, -205.1173479911695097 ) ) ;
#93356=CARTESIAN_POINT ( 'NONE',  ( 37.39189077831895247, -295.5719075428073666, -282.8976365775211548 ) ) ;
#93357=CARTESIAN_POINT ( 'NONE',  ( -94.29573271656752809, -294.5392684802084773, -321.4642638720558807 ) ) ;
#93358=CARTESIAN_POINT ( 'NONE',  ( -101.0104740308733966, -278.1049622890552087, -234.1714001431494410 ) ) ;
#93359=CARTESIAN_POINT ( 'NONE',  ( -109.1069308216474667, -272.4130725769809942, -242.4786282469997616 ) ) ;
#93360=CARTESIAN_POINT ( 'NONE',  ( 10.72929207825920273, -292.8531278653502454, -326.2170707445384323 ) ) ;
#93361=CARTESIAN_POINT ( 'NONE',  ( 8.221610683803218578, -278.1796416044845159, -328.7527519124992637 ) ) ;
#93362=CARTESIAN_POINT ( 'NONE',  ( -49.04723166040062665, -272.0411600202263003, -197.0025594693185553 ) ) ;
#93363=B_SPLINE_CURVE_WITH_KNOTS ( 'NONE', 3,
 ( #43081, #63952, #57763, #92791, #43538, #56849, #7552, #20837, #20378, #87083, #49706, #49249, #13745, #85690, #42594, #86609 ),
 .UNSPECIFIED., .F., .F.,
 ( 4, 2, 2, 2, 2, 2, 2, 4 ),
 ( 0.6790892544725759539, 0.7192030976635021000, 0.7593169408544281351, 0.7994307840453542813, 0.8395446272362804274, 0.8796584704272065736, 0.9197723136181326087, 1.000000000000000000 ),
 .UNSPECIFIED. ) ;
#93364=CARTESIAN_POINT ( 'NONE',  ( 30.96068055187923562, -295.1162384671271184, -297.3687305822743951 ) ) ;
#93365=CARTESIAN_POINT ( 'NONE',  ( -101.7322937367429603, -297.1555027337522006, -305.4050550830162365 ) ) ;
#93367=CARTESIAN_POINT ( 'NONE',  ( -79.57341909547156433, -295.4833137061534103, -208.1172801465939983 ) ) ;
#93368=CARTESIAN_POINT ( 'NONE',  ( -54.58039129470394357, -298.4876434721509213, -195.4202058375244633 ) ) ;
#93369=CARTESIAN_POINT ( 'NONE',  ( 29.95662235446795307, -286.5258288642655202, -300.2584461071188002 ) ) ;
#93370=CARTESIAN_POINT ( 'NONE',  ( -109.8808681630931119, -274.7995226287691253, -251.1073299375090073 ) ) ;
#93371=CARTESIAN_POINT ( 'NONE',  ( -72.46119749723085590, -290.4704361033876694, -334.6264224092256541 ) ) ;
#93372=CARTESIAN_POINT ( 'NONE',  ( -88.00056946223183729, -273.8583572385398384, -212.3834080900900858 ) ) ;
#93373=CARTESIAN_POINT ( 'NONE',  ( -71.67869562670523464, -297.9185484927414791, -205.9026899569780085 ) ) ;
#93374=CARTESIAN_POINT ( 'NONE',  ( -108.9937543560073578, -280.8338736804565201, -246.8631647424808193 ) ) ;
#93375=CARTESIAN_POINT ( 'NONE',  ( 37.50573183366711305, -280.0367153198178585, -254.4503454605764432 ) ) ;
#93377=CARTESIAN_POINT ( 'NONE',  ( -65.22297454738438205, -282.7556847950644396, -342.0408276124356917 ) ) ;
#93378=CARTESIAN_POINT ( 'NONE',  ( 16.87746370896037718, -275.6533848292824587, -324.9661437295197857 ) ) ;
#93379=CARTESIAN_POINT ( 'NONE',  ( -19.91912720295708183, -278.6722086477174685, -196.1254167293053001 ) ) ;
#93380=CARTESIAN_POINT ( 'NONE',  ( -53.34471614677429585, -277.8473460212447321, -196.8644592883882751 ) ) ;
#93381=CARTESIAN_POINT ( 'NONE',  ( -109.7057917503941837, -271.3054263375146320, -256.7167939506281868 ) ) ;
#93382=CARTESIAN_POINT ( 'NONE',  ( 19.54902106401569029, -278.2297495938773864, -319.2522849109691379 ) ) ;
#93384=CARTESIAN_POINT ( 'NONE',  ( 25.14345832407315839, -291.0041463908388550, -228.1502657429280134 ) ) ;
#93385=CARTESIAN_POINT ( 'NONE',  ( -106.0041104324170220, -291.0021413791034774, -235.3942584584674762 ) ) ;
#93386=CARTESIAN_POINT ( 'NONE',  ( 27.52695381552508991, -278.0586348456372434, -308.3359275282518297 ) ) ;
#93387=CARTESIAN_POINT ( 'NONE',  ( -109.1029005865617307, -270.8350489111158481, -248.3813384008189757 ) ) ;
#93388=CARTESIAN_POINT ( 'NONE',  ( -33.72468060359333464, -285.2937548822400800, -193.6077728402057403 ) ) ;
#93391=CARTESIAN_POINT ( 'NONE',  ( -97.91278823630773331, -283.1550164924902333, -226.1114543003701840 ) ) ;
#93393=CARTESIAN_POINT ( 'NONE',  ( 35.81900950809895079, -292.4242918366943513, -276.2467844365119731 ) ) ;
#93394=CARTESIAN_POINT ( 'NONE',  ( 32.13892928045079600, -285.3470132185835269, -244.0757299866895664 ) ) ;
#93397=CARTESIAN_POINT ( 'NONE',  ( -74.30981107682269737, -293.5435474178731852, -335.6172243832690469 ) ) ;
#93398=CARTESIAN_POINT ( 'NONE',  ( -102.3377423507916859, -282.5047976998575905, -310.3388898952244972 ) ) ;
#93399=CARTESIAN_POINT ( 'NONE',  ( -102.8755574070748793, -280.6101255035393933, -236.3123390918978544 ) ) ;
#93400=CARTESIAN_POINT ( 'NONE',  ( -35.17492549822232917, -287.2838279302326328, -193.7757638536210720 ) ) ;
#93401=CARTESIAN_POINT ( 'NONE',  ( -1.592100343325223877, -278.7592742957497762, -203.3093459649720671 ) ) ;
#93402=CARTESIAN_POINT ( 'NONE',  ( 29.42505706653262365, -287.9508718134921423, -300.0026327109038675 ) ) ;
#93403=CARTESIAN_POINT ( 'NONE',  ( -71.91508889801768589, -278.9438669585422303, -335.3372857805192666 ) ) ;
#93404=CARTESIAN_POINT ( 'NONE',  ( -103.2721016708898532, -278.9254593197376266, -302.1924037059603165 ) ) ;
#93405=CARTESIAN_POINT ( 'NONE',  ( -107.5064108168476338, -286.8896419441156240, -242.7359989365525905 ) ) ;
#93407=CARTESIAN_POINT ( 'NONE',  ( -37.60553200451163747, -297.8822550093572659, -193.3615699496105265 ) ) ;
#93408=CARTESIAN_POINT ( 'NONE',  ( 34.67537222130464869, -289.7879136342854736, -290.1844754086752687 ) ) ;
#93410=CARTESIAN_POINT ( 'NONE',  ( -37.30987171927208124, -285.5519495502701375, -350.3611179825600175 ) ) ;
#93411=ORIENTED_EDGE ( 'NONE', *, *, #3118, .T. ) ;
#93412=CARTESIAN_POINT ( 'NONE',  ( -31.37946563810588430, -272.1270991627338276, -195.4183176735483016 ) ) ;
#93413=CARTESIAN_POINT ( 'NONE',  ( 19.79250794923519052, -291.2619682345053320, -219.9219310330756230 ) ) ;
#93414=CARTESIAN_POINT ( 'NONE',  ( -66.08311528030476723, -294.9464099139960354, -337.5319412381646202 ) ) ;
#93415=CARTESIAN_POINT ( 'NONE',  ( -6.746146657060896779, -287.9813622172252963, -203.3053366861183520 ) ) ;
#93416=CARTESIAN_POINT ( 'NONE',  ( -6.365495103167028823, -282.2248403249021749, -203.1278769479647224 ) ) ;
#93417=CARTESIAN_POINT ( 'NONE',  ( -4.569199117443258018, -290.0540774315262524, -339.4013495191113634 ) ) ;
#93418=CARTESIAN_POINT ( 'NONE',  ( -29.01410460794515700, -290.2640079778120707, -346.4665827955946042 ) ) ;
#93419=CARTESIAN_POINT ( 'NONE',  ( -90.28865002906135828, -285.8008580650235899, -323.5529205773983108 ) ) ;
#93420=CARTESIAN_POINT ( 'NONE',  ( -71.56894305999588823, -277.6585219453281184, -339.3357208869135206 ) ) ;
#93422=CARTESIAN_POINT ( 'NONE',  ( 36.93707770848498484, -291.8094766409882936, -284.2864993430272307 ) ) ;
#93423=CARTESIAN_POINT ( 'NONE',  ( 3.823765122875361300, -280.4229418822373532, -205.2258335575434103 ) ) ;
#93424=CARTESIAN_POINT ( 'NONE',  ( -109.1407697003461124, -274.6598007323320871, -251.3021906120513904 ) ) ;
#93425=CARTESIAN_POINT ( 'NONE',  ( -4.829096099716510437, -294.9805209788416391, -202.7746430608542312 ) ) ;
#93426=CARTESIAN_POINT ( 'NONE',  ( 16.22477106298412508, -274.5448354871925858, -324.3289756100926411 ) ) ;
#93428=CARTESIAN_POINT ( 'NONE',  ( -43.75024467819104501, -279.4767736568892360, -197.5309062623671252 ) ) ;
#93429=CARTESIAN_POINT ( 'NONE',  ( 35.68873695956158798, -277.0493261069672712, -293.4817576209982235 ) ) ;
#93430=CARTESIAN_POINT ( 'NONE',  ( -36.49290927759641789, -299.4882554922018016, -196.7716739771189793 ) ) ;
#93431=CARTESIAN_POINT ( 'NONE',  ( -18.98631019523740804, -281.8803485584491000, -344.9538147036035411 ) ) ;
#93432=CARTESIAN_POINT ( 'NONE',  ( -102.0199626533828337, -292.7987792331045966, -234.2739070329792810 ) ) ;
#93433=CARTESIAN_POINT ( 'NONE',  ( -69.80961249357252996, -275.2319125000711892, -201.4101059853202855 ) ) ;
#93434=CARTESIAN_POINT ( 'NONE',  ( -58.00463181270065149, -275.1059523535773224, -196.6423389768230265 ) ) ;
#93435=CARTESIAN_POINT ( 'NONE',  ( 37.45292602031227602, -295.5213466841288437, -267.9543934762687059 ) ) ;
#93436=CARTESIAN_POINT ( 'NONE',  ( -48.62974823152696757, -281.1960574144940210, -344.3381981781935792 ) ) ;
#93437=CARTESIAN_POINT ( 'NONE',  ( -112.8480888415426762, -290.0305856769971342, -285.4122601950525677 ) ) ;
#93438=CARTESIAN_POINT ( 'NONE',  ( 35.99407092260890551, -273.3927036144502267, -256.4430904783872620 ) ) ;
#93439=CARTESIAN_POINT ( 'NONE',  ( -33.78526479030544039, -287.6963276090850741, -194.2441541422848275 ) ) ;
#93440=CARTESIAN_POINT ( 'NONE',  ( -109.4855542413283160, -289.3014611403405070, -283.3799653929628448 ) ) ;
#93442=CARTESIAN_POINT ( 'NONE',  ( -101.1816048158095072, -289.6842194989674795, -228.2772408569960874 ) ) ;
#93443=CARTESIAN_POINT ( 'NONE',  ( -97.36870871009104178, -289.6394715030056659, -311.9624778839516352 ) ) ;
#93445=CARTESIAN_POINT ( 'NONE',  ( -3.637656833744716156, -287.5661836699939045, -201.4588427515063813 ) ) ;
#93446=CARTESIAN_POINT ( 'NONE',  ( -74.02022723481208288, -277.8872971944346659, -333.5020170581052525 ) ) ;
#93447=CARTESIAN_POINT ( 'NONE',  ( -4.723082304384085717, -291.3921507254633525, -200.9527735095904291 ) ) ;
#93448=CARTESIAN_POINT ( 'NONE',  ( -96.18694882895684373, -284.5358883346564767, -319.8845140957773765 ) ) ;
#93449=CARTESIAN_POINT ( 'NONE',  ( -113.5778257278640950, -284.7472744917134833, -281.4050597008513819 ) ) ;
#93450=CARTESIAN_POINT ( 'NONE',  ( -5.553124193766756811, -280.8155175398274537, -204.6224389043356382 ) ) ;
#93451=CARTESIAN_POINT ( 'NONE',  ( -113.8400438337849607, -273.7182392849545067, -284.1715810343901580 ) ) ;
#93452=CARTESIAN_POINT ( 'NONE',  ( 184.2263671677063712, 263.6655576831765870, -152.9503626755218590 ) ) ;
#93453=CARTESIAN_POINT ( 'NONE',  ( 183.3501064672990992, 261.6236131564620564, -151.2791749291968415 ) ) ;
#93454=CARTESIAN_POINT ( 'NONE',  ( -54.23893091208370265, -273.0266867937696702, -199.1776555895956733 ) ) ;
#93455=CARTESIAN_POINT ( 'NONE',  ( -24.52894948609698744, -273.1397102019383851, -198.1285675201764604 ) ) ;
#93456=CARTESIAN_POINT ( 'NONE',  ( -8.416994874107269098, -294.1912886284904971, -341.7119300439276230 ) ) ;
#93457=CARTESIAN_POINT ( 'NONE',  ( 199.6417264645343721, 285.7069599252702119, -96.38872539580104615 ) ) ;
#93459=CARTESIAN_POINT ( 'NONE',  ( -85.48484136407371636, -272.0869869860615609, -210.9007427453300068 ) ) ;
#93460=CARTESIAN_POINT ( 'NONE',  ( -71.04922905380782083, -299.4629144823082925, -204.2056963206571254 ) ) ;
#93462=CARTESIAN_POINT ( 'NONE',  ( -23.67716697703319539, -290.1891895229061333, -342.6248294923580602 ) ) ;
#93463=CARTESIAN_POINT ( 'NONE',  ( -28.08087035673225884, -293.2519975431939088, -197.5883353551120649 ) ) ;
#93465=CARTESIAN_POINT ( 'NONE',  ( -95.40103107510299196, -298.1745132989731815, -220.0629045682121330 ) ) ;
#93466=CARTESIAN_POINT ( 'NONE',  ( -44.03625157419021718, -286.4575748318908950, -197.6069330679039808 ) ) ;
#93467=CARTESIAN_POINT ( 'NONE',  ( 34.30462442122028222, -294.7074852069557664, -298.1273384436191805 ) ) ;
#93468=CARTESIAN_POINT ( 'NONE',  ( -32.01050979066527447, -295.4789650893886801, -347.1278980988841454 ) ) ;
#93469=CARTESIAN_POINT ( 'NONE',  ( 35.70799734060722130, -293.7240662909975981, -270.7578046560553844 ) ) ;
#93471=CARTESIAN_POINT ( 'NONE',  ( -49.51186359494247569, -275.8184430987686824, -195.7348543296051560 ) ) ;
#93473=CARTESIAN_POINT ( 'NONE',  ( -113.0062548877486819, -277.8843872511916402, -284.3763473865262199 ) ) ;
#93475=CARTESIAN_POINT ( 'NONE',  ( -24.43672847221546363, -272.6193369866017520, -197.6460266796819667 ) ) ;
#93476=CARTESIAN_POINT ( 'NONE',  ( -34.47575232296714631, -299.2938913470392208, -196.9634389370661438 ) ) ;
#93477=CARTESIAN_POINT ( 'NONE',  ( 20.86125389797872387, -275.8700475353944626, -225.8902316055917368 ) ) ;
#93478=CARTESIAN_POINT ( 'NONE',  ( 1.875567058276114585, -276.3294536600010360, -205.2767114963382085 ) ) ;
#93479=CARTESIAN_POINT ( 'NONE',  ( 4.927374798749446505, -274.5041390199899070, -332.7448667114337582 ) ) ;
#93480=CARTESIAN_POINT ( 'NONE',  ( -23.49140382440393182, -295.5219606246382682, -342.1906606054416216 ) ) ;
#93481=CARTESIAN_POINT ( 'NONE',  ( 10.66227604733319900, -292.9479622675751784, -326.1373959769626936 ) ) ;
#93483=CARTESIAN_POINT ( 'NONE',  ( -113.9831947762480411, -279.1363068300817645, -263.0260339418780973 ) ) ;
#93484=CARTESIAN_POINT ( 'NONE',  ( -27.01941584524472617, -277.0839261023417635, -342.6276417101828997 ) ) ;
#93485=CARTESIAN_POINT ( 'NONE',  ( -52.06188809211826651, -284.5524896018435470, -195.2296895823323268 ) ) ;
#93486=CARTESIAN_POINT ( 'NONE',  ( -95.93368542694700807, -299.1986782260334508, -223.2760068522333938 ) ) ;
#93487=CARTESIAN_POINT ( 'NONE',  ( 82.63238957975535470, -300.8510545236958365, -197.5047496147394668 ) ) ;
#93488=CARTESIAN_POINT ( 'NONE',  ( 18.79221964301244796, -286.0846147172247811, -223.4205486067389472 ) ) ;
#93489=CARTESIAN_POINT ( 'NONE',  ( -30.14180374065835721, -278.3842034294286805, -196.6477564345687483 ) ) ;
#93490=CARTESIAN_POINT ( 'NONE',  ( -108.1806289176360139, -277.3887685684745179, -250.3840498241575858 ) ) ;
#93491=CARTESIAN_POINT ( 'NONE',  ( -101.3259944083016251, -286.0264186511553248, -309.5874242818709376 ) ) ;
#93492=CARTESIAN_POINT ( 'NONE',  ( -16.25217542377819058, -277.9785904355476305, -340.7163565289692428 ) ) ;
#93494=CARTESIAN_POINT ( 'NONE',  ( 19.45336154821961117, -273.2551532189198156, -219.4823559655316387 ) ) ;
#93495=CARTESIAN_POINT ( 'NONE',  ( 19.07223262217143400, -275.5456024874844161, -223.8706796087952284 ) ) ;
#93496=CARTESIAN_POINT ( 'NONE',  ( 24.43838321705250394, -284.1319473700785920, -313.2002312222252272 ) ) ;
#93498=CARTESIAN_POINT ( 'NONE',  ( 36.60903307437060761, -289.2738158650947753, -254.7871740450747780 ) ) ;
#93499=CARTESIAN_POINT ( 'NONE',  ( 31.14616550503944481, -291.9540899036791757, -301.0551009103980391 ) ) ;
#93500=CARTESIAN_POINT ( 'NONE',  ( 15.81498358983247243, -273.5091739102238080, -219.5369595236599025 ) ) ;
#93501=CARTESIAN_POINT ( 'NONE',  ( 7.439904419314146367, -290.8098961646625753, -211.1540797886869427 ) ) ;
#93502=CARTESIAN_POINT ( 'NONE',  ( 9.093980818847771985, -59.61193948127866094, -357.4272672779520121 ) ) ;
#93504=CARTESIAN_POINT ( 'NONE',  ( -89.03612589067078886, -288.2433002536640743, -326.4894895635828220 ) ) ;
#93505=CARTESIAN_POINT ( 'NONE',  ( 37.11086761422676261, -285.9845440276463364, -285.5528648548295223 ) ) ;
#93506=CARTESIAN_POINT ( 'NONE',  ( -33.44703475892746525, -284.4274772773545692, -343.8598892607020616 ) ) ;
#93507=CARTESIAN_POINT ( 'NONE',  ( -70.27848341858285153, -284.3005485007004722, -335.7032985130510951 ) ) ;
#93508=CARTESIAN_POINT ( 'NONE',  ( -111.5565891034642618, -292.6989374988067993, -257.3013684094283349 ) ) ;
#93509=CARTESIAN_POINT ( 'NONE',  ( -13.07317647120376236, -274.6923430022641810, -197.3078288643833673 ) ) ;
#93510=CARTESIAN_POINT ( 'NONE',  ( -111.7202454524117599, -288.4614405482430470, -283.7439582797645699 ) ) ;
#93511=CARTESIAN_POINT ( 'NONE',  ( -65.09507202992548969, -277.4047905908148550, -342.2418452433019525 ) ) ;
#93512=CARTESIAN_POINT ( 'NONE',  ( 36.09695971889733102, -295.3587144492655057, -256.9256658754217710 ) ) ;
#93514=CARTESIAN_POINT ( 'NONE',  ( -37.37352853689063892, -300.5519495502701943, -195.3611179825600175 ) ) ;
#93515=CARTESIAN_POINT ( 'NONE',  ( -108.5019930357738929, -283.4778503710252267, -251.9911372384626702 ) ) ;
#93516=CARTESIAN_POINT ( 'NONE',  ( -83.32021553195014008, -277.4224509290582432, -211.0419171283040498 ) ) ;
#93517=CARTESIAN_POINT ( 'NONE',  ( -20.70664710831266575, -296.6570049833844109, -194.1655527349372790 ) ) ;
#93518=CARTESIAN_POINT ( 'NONE',  ( 32.61152168340876045, -275.1818891360526322, -291.6280526748131479 ) ) ;
#93519=CARTESIAN_POINT ( 'NONE',  ( 34.62271883042186715, -294.8641433517653354, -254.4336790149428964 ) ) ;
#93520=CARTESIAN_POINT ( 'NONE',  ( 19.52092451065522738, -293.8422999169034711, -224.1888196464184091 ) ) ;
#93521=CARTESIAN_POINT ( 'NONE',  ( -79.19310707031579000, -296.9194207817747611, -334.4060866286340001 ) ) ;
#93522=CARTESIAN_POINT ( 'NONE',  ( -102.5313784318425547, -296.8327218276427857, -237.3957819845661845 ) ) ;
#93523=CARTESIAN_POINT ( 'NONE',  ( -104.6288388657776096, -292.1153715057439513, -303.4887741950014970 ) ) ;
#93524=CARTESIAN_POINT ( 'NONE',  ( -35.89706682933255877, -283.2012159406257297, -347.3606820246671987 ) ) ;
#93525=CARTESIAN_POINT ( 'NONE',  ( -24.34776320107464542, -272.3557753154875058, -195.6655839070433842 ) ) ;
#93526=CARTESIAN_POINT ( 'NONE',  ( -23.78381967985747281, -286.0539782724353017, -194.5099096889770749 ) ) ;
#93527=CARTESIAN_POINT ( 'NONE',  ( -13.23078674303616786, -278.7174624458370431, -341.0590070258358537 ) ) ;
#93528=CARTESIAN_POINT ( 'NONE',  ( -60.04021353905203995, -284.8093570205584228, -200.7322020304045793 ) ) ;
#93530=CARTESIAN_POINT ( 'NONE',  ( -69.79726493871461912, -287.4792636347085590, -337.9891108120561967 ) ) ;
#93531=CARTESIAN_POINT ( 'NONE',  ( -96.00709874043252512, -235.9016261432062720, -336.2420922186948928 ) ) ;
#93532=CARTESIAN_POINT ( 'NONE',  ( -44.02376733478919135, -285.4730392650935187, -197.6057853978923902 ) ) ;
#93533=CARTESIAN_POINT ( 'NONE',  ( 38.39974831866283012, -282.6088882822317032, -258.5614584936393499 ) ) ;
#93534=CARTESIAN_POINT ( 'NONE',  ( -46.01114062161299501, -288.2181544786747622, -346.6876758869118476 ) ) ;
#93535=CARTESIAN_POINT ( 'NONE',  ( -111.3142789937868287, -280.3840882004795390, -252.0182382870230811 ) ) ;
#93536=CARTESIAN_POINT ( 'NONE',  ( -107.1194078006392090, -279.4625646259284508, -301.8646329476553092 ) ) ;
#93537=CARTESIAN_POINT ( 'NONE',  ( -97.99242448250743109, -278.9508199391234484, -229.6451445622688823 ) ) ;
#93538=CARTESIAN_POINT ( 'NONE',  ( -86.40994850451242826, -275.3472863608535590, -214.0413950332018089 ) ) ;
#93539=CARTESIAN_POINT ( 'NONE',  ( 29.57466943630001310, -294.0480726856487195, -308.5634403922383626 ) ) ;
#93540=CARTESIAN_POINT ( 'NONE',  ( -26.25494551295901147, -286.9305839336622057, -344.2301885035767555 ) ) ;
#93541=CARTESIAN_POINT ( 'NONE',  ( -11.44450386862733815, -293.9839521229195043, -198.6413428907675041 ) ) ;
#93542=CARTESIAN_POINT ( 'NONE',  ( -110.1130621978689987, -295.3507015472331432, -279.6313503302699814 ) ) ;
#93543=CARTESIAN_POINT ( 'NONE',  ( 32.71801444650724733, -283.8026522964962624, -295.6721755190951058 ) ) ;
#93544=CARTESIAN_POINT ( 'NONE',  ( -90.42552444425373892, -295.4961676496943710, -320.5756916301675687 ) ) ;
#93545=CARTESIAN_POINT ( 'NONE',  ( -30.73764706975871519, -293.2133162436821863, -193.9025573788531744 ) ) ;
#93546=CARTESIAN_POINT ( 'NONE',  ( -14.28458138705839353, -281.0104726537849729, -200.9371374457803654 ) ) ;
#93548=CARTESIAN_POINT ( 'NONE',  ( 38.69277641733815187, -274.4783923215439927, -259.7980412844152056 ) ) ;
#93549=CARTESIAN_POINT ( 'NONE',  ( -109.7667428805340819, -290.8751381530061053, -296.3631973658353331 ) ) ;
#93550=CARTESIAN_POINT ( 'NONE',  ( -73.70433059592032521, -281.6687339992516286, -336.8881869333473560 ) ) ;
#93551=CARTESIAN_POINT ( 'NONE',  ( -102.2811402926141682, -290.3423449120315922, -311.7945792808152419 ) ) ;
#93552=CARTESIAN_POINT ( 'NONE',  ( -10.71243403179295939, -289.0284593315242887, -338.4077746162614631 ) ) ;
#93554=CARTESIAN_POINT ( 'NONE',  ( 183.3530210459282443, 262.9716507355972226, -152.1700128130211453 ) ) ;
#93555=CARTESIAN_POINT ( 'NONE',  ( 184.7455544834175498, 260.4446745686637996, -151.0159784568642181 ) ) ;
#93556=CARTESIAN_POINT ( 'NONE',  ( 35.78497577281001440, -272.8380690714490129, -253.7030783399848985 ) ) ;
#93557=CARTESIAN_POINT ( 'NONE',  ( -108.9248828707205945, -277.5503714635711390, -285.4756697762999238 ) ) ;
#93558=ORIENTED_EDGE ( 'NONE', *, *, #18309, .T. ) ;
#93559=CARTESIAN_POINT ( 'NONE',  ( -32.93073481843851624, -279.0293548781060622, -197.1848277031661212 ) ) ;
#93560=CARTESIAN_POINT ( 'NONE',  ( 1.188515487324648179, -274.2186665256807032, -203.7037570244632150 ) ) ;
#93561=CARTESIAN_POINT ( 'NONE',  ( 181.1745638653161166, 251.2302727232378459, -164.9768912459212231 ) ) ;
#93563=CARTESIAN_POINT ( 'NONE',  ( -61.84139018168271917, -278.3147013432948143, -197.9287258956971698 ) ) ;
#93564=CARTESIAN_POINT ( 'NONE',  ( -94.70183077768534474, -281.9094567301834218, -318.1278660185766398 ) ) ;
#93565=CARTESIAN_POINT ( 'NONE',  ( -102.2383502863162335, -297.7892401747529902, -309.8883087576965636 ) ) ;
#93566=CARTESIAN_POINT ( 'NONE',  ( -44.31231391334680580, -292.4541006233025655, -197.5820026341282585 ) ) ;
#93567=CARTESIAN_POINT ( 'NONE',  ( -73.80408897849801519, -288.2319407430913998, -334.1857974708884171 ) ) ;
#93568=CARTESIAN_POINT ( 'NONE',  ( -52.53361257456068500, -274.5140145890978260, -194.9242658959265384 ) ) ;
#93569=CARTESIAN_POINT ( 'NONE',  ( -110.1887733950832740, -272.6240159247767565, -264.9134524955282473 ) ) ;
#93573=CARTESIAN_POINT ( 'NONE',  ( -76.76251448157525203, -281.4493582783108536, -205.8388142303484472 ) ) ;
#93575=CARTESIAN_POINT ( 'NONE',  ( 0.5479901314351166564, -281.6493363018157652, -207.5441151669947146 ) ) ;
#93576=CARTESIAN_POINT ( 'NONE',  ( -68.28073092407900901, -281.4114967859224521, -200.9441068037826881 ) ) ;
#93577=CARTESIAN_POINT ( 'NONE',  ( -107.6210902219983012, -283.3387477574189006, -291.0024175355258649 ) ) ;
#93578=CARTESIAN_POINT ( 'NONE',  ( -92.22573883598570887, -281.1173658121962262, -220.3750421590519579 ) ) ;
#93579=CARTESIAN_POINT ( 'NONE',  ( 13.99337936448623765, -273.2685805253104263, -217.4894113236656494 ) ) ;
#93582=CARTESIAN_POINT ( 'NONE',  ( -80.12776709747809889, -278.4178555617960455, -334.2492284253174262 ) ) ;
#93584=CARTESIAN_POINT ( 'NONE',  ( -101.6112971142877228, -276.5793788903895347, -311.7859623163165566 ) ) ;
#93587=CARTESIAN_POINT ( 'NONE',  ( -112.7089963026202213, -286.5006084235405979, -272.8212396622769802 ) ) ;
#93588=CARTESIAN_POINT ( 'NONE',  ( 19.47765081189507796, -292.0984976963708846, -224.2526565087588040 ) ) ;
#93589=CARTESIAN_POINT ( 'NONE',  ( -41.76299922752258453, -288.4550388337621030, -347.1451823561020547 ) ) ;
#93590=CARTESIAN_POINT ( 'NONE',  ( -75.21971805218852580, -283.7796658139261012, -206.7747218624123491 ) ) ;
#93591=CARTESIAN_POINT ( 'NONE',  ( -107.0849701354215853, -283.4381525016597720, -246.7229376067209046 ) ) ;
#93592=CARTESIAN_POINT ( 'NONE',  ( -10.37550522456752589, -286.9353747170914630, -339.3421142969108928 ) ) ;
#93594=CARTESIAN_POINT ( 'NONE',  ( 17.91385157906054459, -283.4427727952519263, -318.6721365095476131 ) ) ;
#93595=CARTESIAN_POINT ( 'NONE',  ( -31.39262931469024309, -272.1270991631888023, -195.5844924281386454 ) ) ;
#93596=CARTESIAN_POINT ( 'NONE',  ( -108.5625833425994671, -282.6038184874507238, -297.6011734199836383 ) ) ;
#93597=CARTESIAN_POINT ( 'NONE',  ( -60.93753984951238323, -297.3584137191123773, -341.6069532050947259 ) ) ;
#93598=CARTESIAN_POINT ( 'NONE',  ( -75.16171495335872521, -283.5496724862859423, -205.3421655673130601 ) ) ;
#93599=CARTESIAN_POINT ( 'NONE',  ( -110.6273434298098266, -279.4895994765356022, -270.6509087954026427 ) ) ;
#93600=CARTESIAN_POINT ( 'NONE',  ( 1.764922937458136332, -288.5741197336049026, -206.1684357019360334 ) ) ;
#93603=CARTESIAN_POINT ( 'NONE',  ( 36.64677586122595443, -295.2761136007291043, -254.9674509712834833 ) ) ;
#93604=CARTESIAN_POINT ( 'NONE',  ( -90.52144297317749988, -275.8047274809828195, -323.3207650710338612 ) ) ;
#93605=CARTESIAN_POINT ( 'NONE',  ( -111.3891023459625131, -289.4916786962212427, -290.8828392937712692 ) ) ;
#93606=CARTESIAN_POINT ( 'NONE',  ( 19.43566057468966335, -292.6134984156360019, -317.5073980996139653 ) ) ;
#93607=CARTESIAN_POINT ( 'NONE',  ( -11.55452602452397315, -279.0798611649137229, -201.4867654609975887 ) ) ;
#93608=CARTESIAN_POINT ( 'NONE',  ( -52.87073974470489190, -295.9907456324371537, -197.7155592323510973 ) ) ;
#93609=CARTESIAN_POINT ( 'NONE',  ( -36.21525922393722396, -293.3817071330117869, -196.8640374757170832 ) ) ;
#93610=CARTESIAN_POINT ( 'NONE',  ( -112.3452863284742875, -275.1604526064900824, -261.9424758988611188 ) ) ;
#93611=CARTESIAN_POINT ( 'NONE',  ( -69.25574402688238251, -293.9442954969541120, -339.6877709368006890 ) ) ;
#93612=CARTESIAN_POINT ( 'NONE',  ( -70.31173089497112016, -291.0942414483819789, -336.4010115599982669 ) ) ;
#93613=CARTESIAN_POINT ( 'NONE',  ( -19.60130737881473806, -290.5169698961747713, -196.4202586060822000 ) ) ;
#93614=CARTESIAN_POINT ( 'NONE',  ( 12.56865776422130843, -289.7657184070116045, -324.5074625283646128 ) ) ;
#93616=CARTESIAN_POINT ( 'NONE',  ( -48.07459332465964508, -289.9948883152570147, -342.7821819764636757 ) ) ;
#93618=CARTESIAN_POINT ( 'NONE',  ( -111.8727705987133305, -291.5340632731458754, -288.1126271521189892 ) ) ;
#93619=CARTESIAN_POINT ( 'NONE',  ( 24.56438554161436372, -280.1525372114587640, -313.3494081264094007 ) ) ;
#93620=CARTESIAN_POINT ( 'NONE',  ( -66.56407526866374269, -291.6584072887602588, -203.4652826028963091 ) ) ;
#93621=CARTESIAN_POINT ( 'NONE',  ( -108.4947299461938002, -279.2589026792759910, -240.9844156633944010 ) ) ;
#93622=CARTESIAN_POINT ( 'NONE',  ( -5.468148163555649255, -282.3109057271302618, -340.4312327019550253 ) ) ;
#93623=CARTESIAN_POINT ( 'NONE',  ( 31.24396662788716128, -285.9510332028983726, -300.8379671649554439 ) ) ;
#93625=CARTESIAN_POINT ( 'NONE',  ( 36.79836970385022710, -279.7404666801557482, -274.1181810831028542 ) ) ;
#93626=CARTESIAN_POINT ( 'NONE',  ( -112.2135809361196408, -282.4853212611050139, -275.5532702530693996 ) ) ;
#93628=CARTESIAN_POINT ( 'NONE',  ( -97.14137382993139624, -277.6721113180604448, -222.9616793681421711 ) ) ;
#93629=CARTESIAN_POINT ( 'NONE',  ( -113.9007273961496196, -283.4056621478234206, -275.6825780289768772 ) ) ;
#93630=CARTESIAN_POINT ( 'NONE',  ( -36.49195868421676892, -299.0043000310293451, -197.1256818783582787 ) ) ;
#93632=CARTESIAN_POINT ( 'NONE',  ( -75.40954654446625227, -293.1359241787627639, -207.0774047863886551 ) ) ;
#93633=CARTESIAN_POINT ( 'NONE',  ( 35.16503031913268273, -276.6696522843807884, -246.0826214834766006 ) ) ;
#93634=CARTESIAN_POINT ( 'NONE',  ( 11.75878309051212511, -276.0147291737525848, -324.4781314715482381 ) ) ;
#93635=CARTESIAN_POINT ( 'NONE',  ( 20.38844535829213811, -296.2132047940258985, -318.2383668027111980 ) ) ;
#93636=CARTESIAN_POINT ( 'NONE',  ( -62.76164968260442123, -289.5406294146090431, -343.1005545414096787 ) ) ;
#93637=CARTESIAN_POINT ( 'NONE',  ( 38.26960366667024260, -279.6269186979536698, -269.9627309050462713 ) ) ;
#93638=CARTESIAN_POINT ( 'NONE',  ( -30.69515346537066591, -291.9671658303655022, -193.5957569260099262 ) ) ;
#93639=CARTESIAN_POINT ( 'NONE',  ( -92.72661084203879511, -290.2914888084347353, -222.4453573829819391 ) ) ;
#93640=CARTESIAN_POINT ( 'NONE',  ( -6.640318923675122775, -292.6488985916901129, -338.7893712419186727 ) ) ;
#93643=CARTESIAN_POINT ( 'NONE',  ( -4.800041469428300012, -292.0003163988286019, -204.9328945002685316 ) ) ;
#93645=CARTESIAN_POINT ( 'NONE',  ( -82.08285599513421005, -270.9094976428775681, -214.2051214447836571 ) ) ;
#93646=CARTESIAN_POINT ( 'NONE',  ( -85.06075887379175526, -296.4703360628379301, -210.2303301555177768 ) ) ;
#93647=CARTESIAN_POINT ( 'NONE',  ( -111.7356591822077974, -285.6418680510804506, -288.2725368821278380 ) ) ;
#93648=CARTESIAN_POINT ( 'NONE',  ( -4.592658239440970291, -286.3294855494381750, -205.1192582611393789 ) ) ;
#93649=CARTESIAN_POINT ( 'NONE',  ( 8.022286106713780285, -277.9396609681482460, -328.5021096233390949 ) ) ;
#93650=CARTESIAN_POINT ( 'NONE',  ( -42.52863166926879046, -293.1380147688722104, -344.8254889573555033 ) ) ;
#93651=CARTESIAN_POINT ( 'NONE',  ( 36.54474554761870309, -295.2454610408362328, -265.2239831728599597 ) ) ;
#93652=CARTESIAN_POINT ( 'NONE',  ( 33.27571837895451523, -274.6106959456377012, -290.4148429090494687 ) ) ;
#93655=CARTESIAN_POINT ( 'NONE',  ( -97.39361016638247293, -295.5731925589939806, -318.5432969909085159 ) ) ;
#93656=CARTESIAN_POINT ( 'NONE',  ( -34.49899005536793339, -290.9364441214599992, -344.7973821129947964 ) ) ;
#93657=CARTESIAN_POINT ( 'NONE',  ( 201.3832976022252694, 295.1831209208456244, -54.00000000002625455 ) ) ;
#93658=CARTESIAN_POINT ( 'NONE',  ( -60.06965241856088511, -298.8441150545593814, -197.0601143195720795 ) ) ;
#93659=CARTESIAN_POINT ( 'NONE',  ( 16.96078226772647568, -287.5035835097140762, -221.4023360966625091 ) ) ;
#93662=CARTESIAN_POINT ( 'NONE',  ( -25.42027612801576808, -279.2593031002447219, -194.5277489276803919 ) ) ;
#93663=CARTESIAN_POINT ( 'NONE',  ( 36.27452867675225434, -294.4849394841311891, -292.7668586998679530 ) ) ;
#93664=CARTESIAN_POINT ( 'NONE',  ( -92.70664402750746547, -287.9743013490632393, -322.1574334306898777 ) ) ;
#93666=CARTESIAN_POINT ( 'NONE',  ( -114.3449454533130734, -296.8590078222697457, -272.4734489240429980 ) ) ;
#93667=CARTESIAN_POINT ( 'NONE',  ( 33.96953537580622395, -293.6774947106861759, -254.5935994513203866 ) ) ;
#93672=CARTESIAN_POINT ( 'NONE',  ( 37.03940563166408850, -288.8566384710205170, -253.2691433512485730 ) ) ;
#93673=CARTESIAN_POINT ( 'NONE',  ( 36.60358173371529489, -284.6237833571632905, -234.7871824221999191 ) ) ;
#93674=CARTESIAN_POINT ( 'NONE',  ( -35.33037011089251678, -279.4253352337865408, -193.4762396088509888 ) ) ;
#93675=CARTESIAN_POINT ( 'NONE',  ( -34.75836376808485539, -285.0198105545406975, -345.1626010497900552 ) ) ;
#93676=CARTESIAN_POINT ( 'NONE',  ( -105.2687266526521341, -282.6710946624464214, -305.4698356563340553 ) ) ;
#93677=CARTESIAN_POINT ( 'NONE',  ( 31.81407040063420055, -285.9950772939433818, -298.0462333479432004 ) ) ;
#93678=CARTESIAN_POINT ( 'NONE',  ( -9.641004424644274096, -278.5544740503940488, -340.8804553185084956 ) ) ;
#93679=CARTESIAN_POINT ( 'NONE',  ( -90.21484266159087895, -273.6116868797454913, -219.9789643280970495 ) ) ;
#93681=CARTESIAN_POINT ( 'NONE',  ( 10.60064419608459119, -293.0580428276577436, -326.0636771462835100 ) ) ;
#93682=CARTESIAN_POINT ( 'NONE',  ( -108.8872461603217374, -278.7442524177691325, -255.7988692541840408 ) ) ;
#93683=CARTESIAN_POINT ( 'NONE',  ( -76.87000942377420643, -278.8563283414132457, -208.8076459835046137 ) ) ;
#93684=CARTESIAN_POINT ( 'NONE',  ( -13.17298574084568941, -275.4386129624982118, -197.5781134136069852 ) ) ;
#93685=CARTESIAN_POINT ( 'NONE',  ( -113.6847796836970446, -277.2601015759275924, -277.2798653054476290 ) ) ;
#93686=CARTESIAN_POINT ( 'NONE',  ( -113.6754805203053849, -271.0251410464779838, -270.3416754731575224 ) ) ;
#93688=CARTESIAN_POINT ( 'NONE',  ( -111.7279744946049931, -297.7565017923008099, -287.8901620553351108 ) ) ;
#93692=CARTESIAN_POINT ( 'NONE',  ( -102.5194722319832437, -286.0860743657551666, -236.8039414588454292 ) ) ;
#93693=CARTESIAN_POINT ( 'NONE',  ( -107.0062009307126516, -286.7057907450686116, -239.8842628368695955 ) ) ;
#93694=CARTESIAN_POINT ( 'NONE',  ( 35.65497047700259969, -286.8378613571862843, -265.5883020783349480 ) ) ;
#93695=CARTESIAN_POINT ( 'NONE',  ( -101.3714150919689843, -283.4968292794517879, -313.1149287536795782 ) ) ;
#93696=CARTESIAN_POINT ( 'NONE',  ( 33.89105063424882758, -279.6993192773426244, -251.0167181872071183 ) ) ;
#93697=CARTESIAN_POINT ( 'NONE',  ( -27.69917805843504510, -288.0363375717602139, -196.7548190202378748 ) ) ;
#93698=CARTESIAN_POINT ( 'NONE',  ( -8.962625000209827775, -278.9100997851881516, -202.3512962782413922 ) ) ;
#93699=CARTESIAN_POINT ( 'NONE',  ( -91.31873723241153584, -279.1550691300693074, -320.3122010175063679 ) ) ;
#93700=CARTESIAN_POINT ( 'NONE',  ( 17.32743406173155876, -275.3517884738028556, -221.8168489556452698 ) ) ;
#93701=CARTESIAN_POINT ( 'NONE',  ( -31.87053940794593743, -287.7796243996576777, -346.8207006490806634 ) ) ;
#93702=CARTESIAN_POINT ( 'NONE',  ( -37.30404601501494000, -283.8544837284365485, -347.2126711055896067 ) ) ;
#93703=CARTESIAN_POINT ( 'NONE',  ( 24.20964569095865215, -282.6593706397758297, -316.5234265393917212 ) ) ;
#93707=CARTESIAN_POINT ( 'NONE',  ( -8.678122513834807705, -290.5414901964716137, -340.5086359251633326 ) ) ;
#93708=CARTESIAN_POINT ( 'NONE',  ( -111.7867486921140312, -289.0142218403041738, -288.0590210152830650 ) ) ;
#93709=CARTESIAN_POINT ( 'NONE',  ( -76.68055102402266243, -272.5700539449761663, -208.5884439425717574 ) ) ;
#93710=CARTESIAN_POINT ( 'NONE',  ( 33.23413576049146911, -292.5111270925425515, -239.8264790471268100 ) ) ;
#93711=CARTESIAN_POINT ( 'NONE',  ( -97.92987621354390626, -288.4528223111061607, -312.3330354371690873 ) ) ;
#93712=CARTESIAN_POINT ( 'NONE',  ( 28.04290555140037355, -292.2593024281230782, -305.1523755245782468 ) ) ;
#93713=CARTESIAN_POINT ( 'NONE',  ( 35.94814091805673684, -288.6940514394966613, -265.5454418533481658 ) ) ;
#93714=CARTESIAN_POINT ( 'NONE',  ( -95.99890600148557951, -299.6948066931273615, -223.6242672951989618 ) ) ;
#93715=CARTESIAN_POINT ( 'NONE',  ( -18.25046875795010948, -280.8060991788453862, -342.9444327182633288 ) ) ;
#93739=COLOUR_RGB('Sky Blue',0.24,0.69,0.87);
#93740=FILL_AREA_STYLE_COLOUR('',#93739);
#93741=FILL_AREA_STYLE('',(#93740));
#93742=SURFACE_STYLE_FILL_AREA(#93741);
#93743=SURFACE_SIDE_STYLE('',(#93742));
#93744=SURFACE_STYLE_USAGE(.BOTH.,#93743);
#93745=PRESENTATION_STYLE_ASSIGNMENT((#93744));
ENDSEC;
END-ISO-10303-21;
